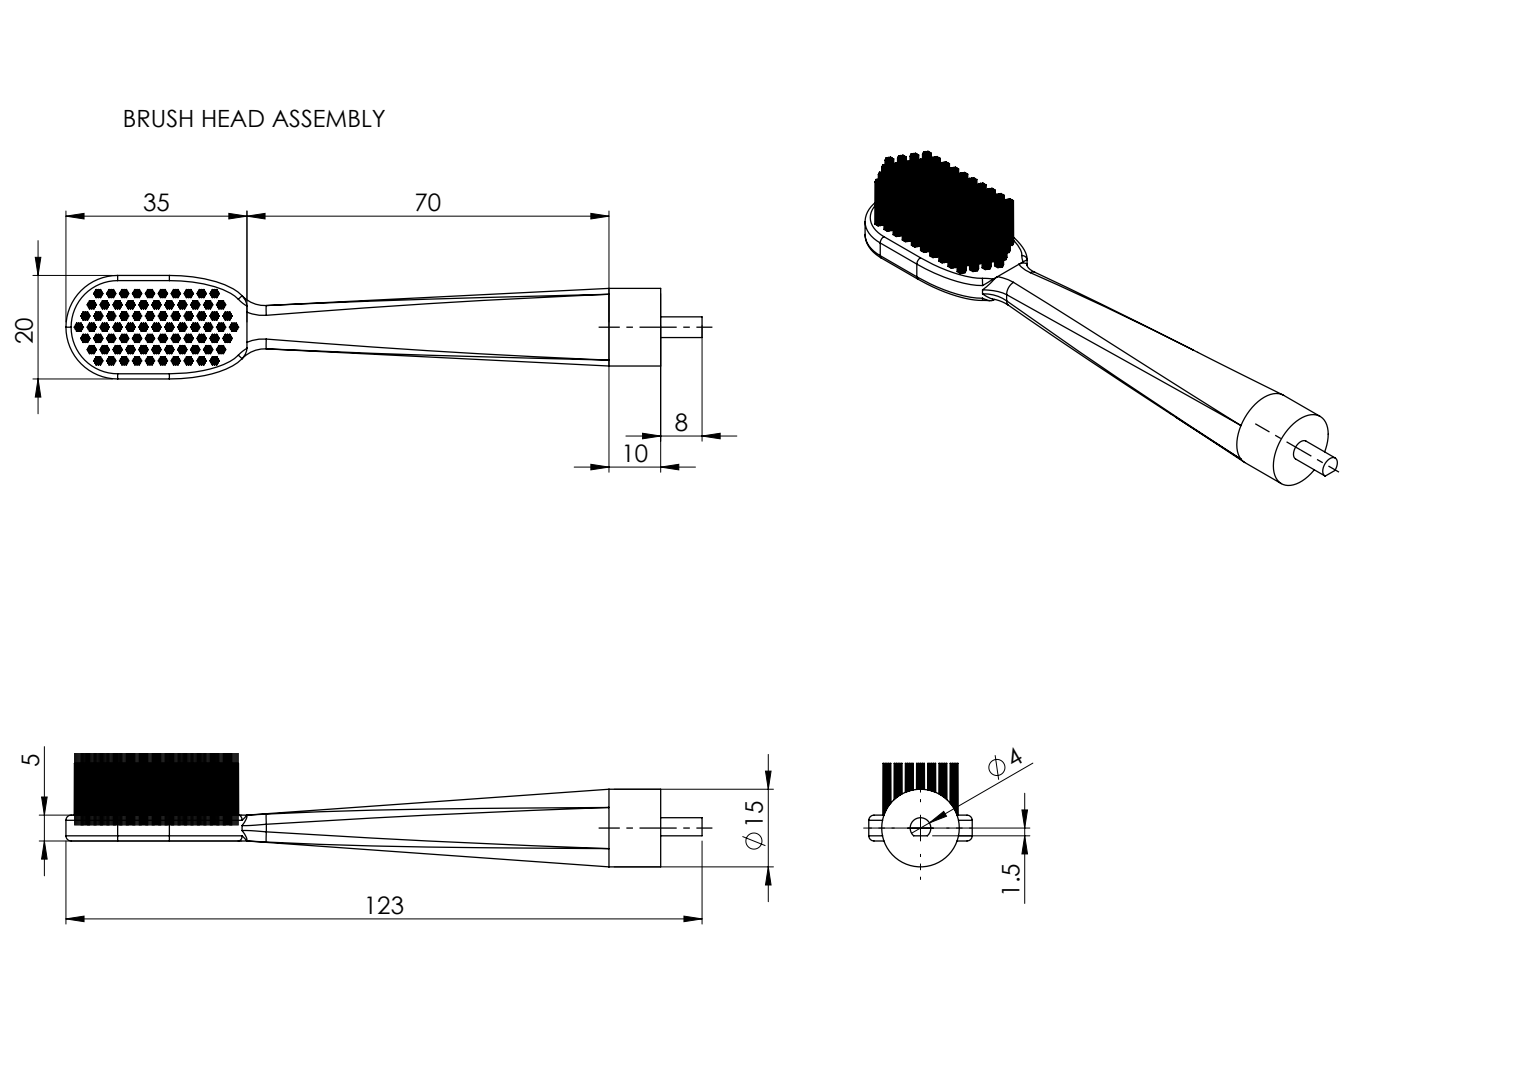
ISO-10303-21;
HEADER;
FILE_DESCRIPTION (('STEP AP214'),
    '1' );
FILE_NAME ('Brush Head Assembly.step',
    '2026-10-02T09:26:43',
    ( '' ),
    ( '' ),
    'SwSTEP 2.0',
    'SolidWorks 2026',
    '' );
FILE_SCHEMA (( 'AUTOMOTIVE_DESIGN' ));
ENDSEC;

DATA;
#1=ORIENTED_EDGE ( 'NONE', *, *, #111289, .F. ) ;
#2=FACE_OUTER_BOUND ( 'NONE', #57861, .T. ) ;
#3=DIRECTION ( 'NONE',  ( 0.000000000000000000, -0.000000000000000000, 1.000000000000000000 ) ) ;
#4=EDGE_CURVE ( 'NONE', #10582, #102432, #129340, .T. ) ;
#6=CIRCLE ( 'NONE', #73182, 0.09999999999999982514 ) ;
#7=CARTESIAN_POINT ( 'NONE',  ( -5.200000000000025935, 12.50000000000000000, -3.983716857408426293 ) ) ;
#8=ADVANCED_FACE ( 'NONE', ( #9369 ), #58491, .T. ) ;
#9=ORIENTED_EDGE ( 'NONE', *, *, #43622, .T. ) ;
#10=DIRECTION ( 'NONE',  ( -0.000000000000000000, 1.000000000000000000, -0.000000000000000000 ) ) ;
#11=AXIS2_PLACEMENT_3D ( 'NONE', #114880, #25207, #65127 ) ;
#12=AXIS2_PLACEMENT_3D ( 'NONE', #43008, #33796, #72443 ) ;
#13=DIRECTION ( 'NONE',  ( 0.000000000000000000, 1.000000000000000000, 0.000000000000000000 ) ) ;
#14=DIRECTION ( 'NONE',  ( 0.000000000000000000, 1.000000000000000000, 0.000000000000000000 ) ) ;
#15=DIRECTION ( 'NONE',  ( 0.000000000000000000, 0.000000000000000000, 1.000000000000000000 ) ) ;
#16=ORIENTED_EDGE ( 'NONE', *, *, #85327, .F. ) ;
#17=ADVANCED_FACE ( 'NONE', ( #79412 ), #68276, .T. ) ;
#18=ORIENTED_EDGE ( 'NONE', *, *, #72941, .T. ) ;
#19=EDGE_CURVE ( 'NONE', #47255, #7520, #102130, .T. ) ;
#20=LINE ( 'NONE', #41902, #103658 ) ;
#21=ORIENTED_EDGE ( 'NONE', *, *, #108659, .T. ) ;
#22=DIRECTION ( 'NONE',  ( 0.000000000000000000, -0.000000000000000000, 1.000000000000000000 ) ) ;
#23=AXIS2_PLACEMENT_3D ( 'NONE', #13282, #3477, #97012 ) ;
#24=CIRCLE ( 'NONE', #104488, 0.1000000000000002554 ) ;
#25=CARTESIAN_POINT ( 'NONE',  ( 17.50000000000000000, -2.499999999999999556, 2.333333333333337478 ) ) ;
#26=DIRECTION ( 'NONE',  ( -0.000000000000000000, -1.000000000000000000, -0.000000000000000000 ) ) ;
#27=VERTEX_POINT ( 'NONE', #38865 ) ;
#28=EDGE_CURVE ( 'NONE', #7615, #17965, #5955, .T. ) ;
#29=CARTESIAN_POINT ( 'NONE',  ( -3.350000000000028511, 2.500000000000000000, -1.472243186433550122 ) ) ;
#30=CARTESIAN_POINT ( 'NONE',  ( 4.549999999999939426, 2.500000000000000000, -6.495190528383302464 ) ) ;
#31=DIRECTION ( 'NONE',  ( 0.000000000000000000, 0.000000000000000000, 1.000000000000000000 ) ) ;
#33=DIRECTION ( 'NONE',  ( 0.000000000000000000, -0.000000000000000000, 1.000000000000000000 ) ) ;
#34=EDGE_CURVE ( 'NONE', #123793, #101138, #123060, .T. ) ;
#35=DIRECTION ( 'NONE',  ( 0.000000000000000000, 0.000000000000000000, 1.000000000000000000 ) ) ;
#36=EDGE_LOOP ( 'NONE', ( #12557, #1627 ) ) ;
#37=ORIENTED_EDGE ( 'NONE', *, *, #25424, .T. ) ;
#38=CARTESIAN_POINT ( 'NONE',  ( -12.09999999999999609, 12.50000000000000000, -3.637306695894647390 ) ) ;
#39=ORIENTED_EDGE ( 'NONE', *, *, #32172, .F. ) ;
#40=DIRECTION ( 'NONE',  ( -0.000000000000000000, 1.000000000000000000, -0.000000000000000000 ) ) ;
#41=ORIENTED_EDGE ( 'NONE', *, *, #63489, .F. ) ;
#42=ORIENTED_EDGE ( 'NONE', *, *, #56795, .T. ) ;
#43=ORIENTED_EDGE ( 'NONE', *, *, #113565, .F. ) ;
#44=CARTESIAN_POINT ( 'NONE',  ( 87.49999999999998579, 2.781865847474100040, -7.000342182495692178 ) ) ;
#45=CIRCLE ( 'NONE', #54416, 0.09999999999999982514 ) ;
#46=CARTESIAN_POINT ( 'NONE',  ( -4.150000000000027889, 12.50000000000000000, -7.253104124594891289 ) ) ;
#47=AXIS2_PLACEMENT_3D ( 'NONE', #50299, #49672, #91507 ) ;
#48=CARTESIAN_POINT ( 'NONE',  ( 10.44999999999991047, 2.500000000000000000, 2.065063509461097624 ) ) ;
#49=CARTESIAN_POINT ( 'NONE',  ( -7.300000000000018474, 12.50000000000000000, 0.3464101615137735735 ) ) ;
#50=DIRECTION ( 'NONE',  ( 0.000000000000000000, -1.000000000000000000, 0.000000000000000000 ) ) ;
#51=DIRECTION ( 'NONE',  ( 0.000000000000000000, 1.000000000000000000, 0.000000000000000000 ) ) ;
#52=CARTESIAN_POINT ( 'NONE',  ( 5.649999999999932854, 2.500000000000000000, 1.918653347947321564 ) ) ;
#53=DIRECTION ( 'NONE',  ( 0.000000000000000000, 0.000000000000000000, 1.000000000000000000 ) ) ;
#54=FACE_OUTER_BOUND ( 'NONE', #43393, .T. ) ;
#55=AXIS2_PLACEMENT_3D ( 'NONE', #102666, #47947, #87846 ) ;
#56=ORIENTED_EDGE ( 'NONE', *, *, #30639, .F. ) ;
#57=ORIENTED_EDGE ( 'NONE', *, *, #57612, .F. ) ;
#58=DIRECTION ( 'NONE',  ( 0.000000000000000000, 0.000000000000000000, -1.000000000000000000 ) ) ;
#59=EDGE_LOOP ( 'NONE', ( #8980, #73677, #9720, #73966 ) ) ;
#60=EDGE_LOOP ( 'NONE', ( #125831, #14201 ) ) ;
#62=CIRCLE ( 'NONE', #54353, 0.09999999999999982514 ) ;
#63=EDGE_CURVE ( 'NONE', #31481, #67997, #18539, .T. ) ;
#64=AXIS2_PLACEMENT_3D ( 'NONE', #6513, #46469, #75933 ) ;
#66=CIRCLE ( 'NONE', #71172, 0.09999999999999982514 ) ;
#67=DIRECTION ( 'NONE',  ( -4.274815082592931898E-19, -0.9999939076577903929, -0.003490651415223739937 ) ) ;
#68=PLANE ( 'NONE',  #922 ) ;
#69=ADVANCED_FACE ( 'NONE', ( #17890 ), #95870, .T. ) ;
#70=DIRECTION ( 'NONE',  ( 0.000000000000000000, -0.9999939076577903929, 0.003490651415223739937 ) ) ;
#71=ORIENTED_EDGE ( 'NONE', *, *, #16257, .F. ) ;
#72=EDGE_CURVE ( 'NONE', #118132, #124753, #125105, .T. ) ;
#73=EDGE_CURVE ( 'NONE', #114203, #127721, #49320, .T. ) ;
#74=AXIS2_PLACEMENT_3D ( 'NONE', #92885, #52954, #31387 ) ;
#75=ADVANCED_FACE ( 'NONE', ( #29656 ), #54076, .T. ) ;
#76=VERTEX_POINT ( 'NONE', #89217 ) ;
#77=PLANE ( 'NONE',  #104864 ) ;
#78=EDGE_LOOP ( 'NONE', ( #93082, #10412 ) ) ;
#79=CARTESIAN_POINT ( 'NONE',  ( 3.549999999999941203, 2.500000000000000000, 6.248780366869521430 ) ) ;
#80=EDGE_CURVE ( 'NONE', #111625, #116591, #38188, .T. ) ;
#81=AXIS2_PLACEMENT_3D ( 'NONE', #66786, #108010, #119130 ) ;
#82=ORIENTED_EDGE ( 'NONE', *, *, #37576, .T. ) ;
#83=ORIENTED_EDGE ( 'NONE', *, *, #49852, .F. ) ;
#84=DIRECTION ( 'NONE',  ( -0.000000000000000000, 1.000000000000000000, -0.000000000000000000 ) ) ;
#85=CARTESIAN_POINT ( 'NONE',  ( -7.100000000000017408, 2.500000000000000000, -4.922947341949753586 ) ) ;
#86=EDGE_CURVE ( 'NONE', #7115, #38409, #127252, .T. ) ;
#87=ADVANCED_FACE ( 'NONE', ( #57833 ), #118026, .T. ) ;
#88=CARTESIAN_POINT ( 'NONE',  ( 13.34999999999990017, 2.500000000000000000, 1.572243186433545548 ) ) ;
#89=DIRECTION ( 'NONE',  ( 0.000000000000000000, 0.000000000000000000, 1.000000000000000000 ) ) ;
#90=CARTESIAN_POINT ( 'NONE',  ( 17.50000000000000000, -2.083333333333333925, 4.000000000000001776 ) ) ;
#91=ORIENTED_EDGE ( 'NONE', *, *, #128566, .T. ) ;
#93=DIRECTION ( 'NONE',  ( -0.000000000000000000, 1.000000000000000000, -0.000000000000000000 ) ) ;
#94=DIRECTION ( 'NONE',  ( -4.274815082592931898E-19, -0.9999939076577903929, -0.003490651415223739937 ) ) ;
#95=CARTESIAN_POINT ( 'NONE',  ( -2.050000000000033129, 2.500000000000000000, 2.165063509461097713 ) ) ;
#96=CARTESIAN_POINT ( 'NONE',  ( -2.950000000000029932, 2.500000000000000000, -2.165063509461101710 ) ) ;
#97=FACE_OUTER_BOUND ( 'NONE', #13668, .T. ) ;
#98=EDGE_LOOP ( 'NONE', ( #5007, #26491, #107521, #16284 ) ) ;
#99=ORIENTED_EDGE ( 'NONE', *, *, #48484, .T. ) ;
#100=CIRCLE ( 'NONE', #16803, 0.06509327318403745899 ) ;
#101=DIRECTION ( 'NONE',  ( 0.000000000000000000, -0.000000000000000000, 1.000000000000000000 ) ) ;
#102=AXIS2_PLACEMENT_3D ( 'NONE', #59335, #77010, #59983 ) ;
#103=ORIENTED_EDGE ( 'NONE', *, *, #8467, .T. ) ;
#104=CARTESIAN_POINT ( 'NONE',  ( 17.41716098457700923, -1.872967139268051806, 4.643356076170615410 ) ) ;
#105=LINE ( 'NONE', #118591, #98263 ) ;
#106=AXIS2_PLACEMENT_3D ( 'NONE', #112814, #42811, #102353 ) ;
#107=VERTEX_POINT ( 'NONE', #106909 ) ;
#108=DIRECTION ( 'NONE',  ( 0.000000000000000000, 1.000000000000000000, 0.000000000000000000 ) ) ;
#109=CARTESIAN_POINT ( 'NONE',  ( -6.650000000000019007, 2.500000000000000000, -5.802370205355749988 ) ) ;
#110=CARTESIAN_POINT ( 'NONE',  ( 10.39999999999991509, 12.50000000000000000, -0.6928203230275542523 ) ) ;
#112=FACE_OUTER_BOUND ( 'NONE', #22375, .T. ) ;
#113=VERTEX_POINT ( 'NONE', #17219 ) ;
#114=DIRECTION ( 'NONE',  ( 0.000000000000000000, -0.9999939076577903929, 0.003490651415223739937 ) ) ;
#115=DIRECTION ( 'NONE',  ( 0.000000000000000000, 0.000000000000000000, 1.000000000000000000 ) ) ;
#116=CARTESIAN_POINT ( 'NONE',  ( -5.200000000000022382, 12.50000000000000000, 0.2813168883297361700 ) ) ;
#117=ADVANCED_FACE ( 'NONE', ( #57173 ), #7419, .T. ) ;
#118=VERTEX_POINT ( 'NONE', #50574 ) ;
#119=DIRECTION ( 'NONE',  ( -0.000000000000000000, 1.000000000000000000, -0.000000000000000000 ) ) ;
#120=EDGE_LOOP ( 'NONE', ( #58165, #15953, #18369, #114695 ) ) ;
#122=DIRECTION ( 'NONE',  ( 0.000000000000000000, -0.000000000000000000, 1.000000000000000000 ) ) ;
#123=DIRECTION ( 'NONE',  ( -4.274815082592931898E-19, -0.9999939076577903929, -0.003490651415223739937 ) ) ;
#124=VERTEX_POINT ( 'NONE', #122556 ) ;
#125=VECTOR ( 'NONE', #104094, 1000.000000000000000 ) ;
#126=CARTESIAN_POINT ( 'NONE',  ( 2.099999999999950351, 12.50000000000000000, -5.022947341949754119 ) ) ;
#127=CONICAL_SURFACE ( 'NONE', #108793, 0.1000000000000000472, 0.003490658503988666988 ) ;
#128=CARTESIAN_POINT ( 'NONE',  ( 1.449999999999951328, 12.50000000000000000, -1.883746621131363597 ) ) ;
#129=EDGE_LOOP ( 'NONE', ( #126937, #8373, #2231, #124616 ) ) ;
#130=CARTESIAN_POINT ( 'NONE',  ( 8.749999999999957367, 2.500000000000000000, -6.595190528383302109 ) ) ;
#131=EDGE_LOOP ( 'NONE', ( #50533, #103161, #4898, #53969 ) ) ;
#132=CONICAL_SURFACE ( 'NONE', #108799, 0.1000000000000002554, 0.003490658503988666988 ) ;
#133=FACE_OUTER_BOUND ( 'NONE', #40974, .T. ) ;
#134=ORIENTED_EDGE ( 'NONE', *, *, #111458, .F. ) ;
#135=DIRECTION ( 'NONE',  ( 0.000000000000000000, 0.000000000000000000, 1.000000000000000000 ) ) ;
#136=CARTESIAN_POINT ( 'NONE',  ( -5.000000000000023093, 2.500000000000000000, 5.022947341949748790 ) ) ;
#137=VERTEX_POINT ( 'NONE', #41429 ) ;
#138=ORIENTED_EDGE ( 'NONE', *, *, #94725, .F. ) ;
#139=DIRECTION ( 'NONE',  ( -0.000000000000000000, 1.000000000000000000, -0.000000000000000000 ) ) ;
#141=ORIENTED_EDGE ( 'NONE', *, *, #10108, .F. ) ;
#142=AXIS2_PLACEMENT_3D ( 'NONE', #9136, #110553, #47778 ) ;
#143=FACE_OUTER_BOUND ( 'NONE', #8076, .T. ) ;
#145=AXIS2_PLACEMENT_3D ( 'NONE', #45558, #95932, #15417 ) ;
#146=DIRECTION ( 'NONE',  ( 0.000000000000000000, 0.000000000000000000, 1.000000000000000000 ) ) ;
#147=CARTESIAN_POINT ( 'NONE',  ( -13.94999999999998685, 12.50000000000000000, -2.576566944158912964 ) ) ;
#148=CARTESIAN_POINT ( 'NONE',  ( -8.300000000000009592, 12.50000000000000000, 4.395220292106234439 ) ) ;
#149=DIRECTION ( 'NONE',  ( 0.000000000000000000, 0.000000000000000000, -1.000000000000000000 ) ) ;
#150=CARTESIAN_POINT ( 'NONE',  ( -0.6500000000000394351, 2.500000000000000000, 6.941600689897073018 ) ) ;
#151=CONICAL_SURFACE ( 'NONE', #75377, 0.09999999999999982514, 0.003490658503988666988 ) ;
#152=EDGE_CURVE ( 'NONE', #35689, #125708, #77064, .T. ) ;
#153=ORIENTED_EDGE ( 'NONE', *, *, #4789, .F. ) ;
#154=ORIENTED_EDGE ( 'NONE', *, *, #109368, .T. ) ;
#155=ORIENTED_EDGE ( 'NONE', *, *, #127999, .F. ) ;
#156=AXIS2_PLACEMENT_3D ( 'NONE', #115565, #16713, #35116 ) ;
#157=CARTESIAN_POINT ( 'NONE',  ( -6.249999999999981348, 12.50000000000000000, 2.165063509461097713 ) ) ;
#158=DIRECTION ( 'NONE',  ( -0.000000000000000000, 1.000000000000000000, -0.000000000000000000 ) ) ;
#159=DIRECTION ( 'NONE',  ( 0.000000000000000000, 0.000000000000000000, 1.000000000000000000 ) ) ;
#160=EDGE_LOOP ( 'NONE', ( #92531, #41100 ) ) ;
#161=EDGE_CURVE ( 'NONE', #53677, #62914, #60358, .T. ) ;
#162=FACE_BOUND ( 'NONE', #99510, .T. ) ;
#163=ORIENTED_EDGE ( 'NONE', *, *, #63007, .F. ) ;
#164=EDGE_CURVE ( 'NONE', #64447, #41921, #37367, .T. ) ;
#165=CARTESIAN_POINT ( 'NONE',  ( -7.900000000000014566, 12.50000000000000000, 0.6277270498435120194 ) ) ;
#166=CARTESIAN_POINT ( 'NONE',  ( 7.899999999999924860, 2.500000000000000000, 5.022947341949748790 ) ) ;
#167=LINE ( 'NONE', #110140, #49263 ) ;
#168=FACE_OUTER_BOUND ( 'NONE', #42884, .T. ) ;
#169=DIRECTION ( 'NONE',  ( -0.000000000000000000, 1.000000000000000000, -0.000000000000000000 ) ) ;
#170=EDGE_CURVE ( 'NONE', #109777, #63696, #31113, .T. ) ;
#171=DIRECTION ( 'NONE',  ( 0.000000000000000000, 1.000000000000000000, 0.000000000000000000 ) ) ;
#172=EDGE_CURVE ( 'NONE', #110736, #16781, #3893, .T. ) ;
#173=DIRECTION ( 'NONE',  ( 0.000000000000000000, 0.000000000000000000, -1.000000000000000000 ) ) ;
#174=EDGE_CURVE ( 'NONE', #53227, #49994, #90490, .T. ) ;
#175=CARTESIAN_POINT ( 'NONE',  ( 11.84999999999990727, 2.500000000000000000, 6.841600689897072485 ) ) ;
#176=ADVANCED_FACE ( 'NONE', ( #101629 ), #14347, .T. ) ;
#177=FACE_OUTER_BOUND ( 'NONE', #72478, .T. ) ;
#178=ORIENTED_EDGE ( 'NONE', *, *, #7339, .F. ) ;
#179=VERTEX_POINT ( 'NONE', #111417 ) ;
#180=VERTEX_POINT ( 'NONE', #20488 ) ;
#181=VERTEX_POINT ( 'NONE', #62977 ) ;
#182=DIRECTION ( 'NONE',  ( 0.000000000000000000, 1.000000000000000000, 0.000000000000000000 ) ) ;
#183=CIRCLE ( 'NONE', #48229, 0.06509327318403741736 ) ;
#184=LINE ( 'NONE', #92445, #36085 ) ;
#185=AXIS2_PLACEMENT_3D ( 'NONE', #74145, #15849, #15191 ) ;
#186=AXIS2_PLACEMENT_3D ( 'NONE', #87460, #107759, #127405 ) ;
#187=EDGE_LOOP ( 'NONE', ( #105520, #67716, #77716, #43576 ) ) ;
#188=ORIENTED_EDGE ( 'NONE', *, *, #84597, .T. ) ;
#189=EDGE_CURVE ( 'NONE', #19176, #5233, #120978, .T. ) ;
#190=ORIENTED_EDGE ( 'NONE', *, *, #82832, .T. ) ;
#191=AXIS2_PLACEMENT_3D ( 'NONE', #50501, #49243, #90414 ) ;
#192=DIRECTION ( 'NONE',  ( -0.000000000000000000, -1.000000000000000000, -0.000000000000000000 ) ) ;
#193=DIRECTION ( 'NONE',  ( 0.000000000000000000, -0.000000000000000000, 1.000000000000000000 ) ) ;
#194=DIRECTION ( 'NONE',  ( -0.000000000000000000, -1.000000000000000000, -0.000000000000000000 ) ) ;
#195=DIRECTION ( 'NONE',  ( 0.000000000000000000, 0.000000000000000000, -1.000000000000000000 ) ) ;
#196=CARTESIAN_POINT ( 'NONE',  ( -8.950000000000004619, 12.50000000000000000, 6.148780366869520897 ) ) ;
#197=CONICAL_SURFACE ( 'NONE', #119337, 0.1000000000000000056, 0.003490658503988666988 ) ;
#198=DIRECTION ( 'NONE',  ( 0.000000000000000000, -0.000000000000000000, 1.000000000000000000 ) ) ;
#199=ORIENTED_EDGE ( 'NONE', *, *, #119327, .F. ) ;
#200=DIRECTION ( 'NONE',  ( 0.000000000000000000, -0.9999939076577903929, 0.003490651415223739937 ) ) ;
#201=ORIENTED_EDGE ( 'NONE', *, *, #13341, .F. ) ;
#202=ORIENTED_EDGE ( 'NONE', *, *, #70316, .F. ) ;
#203=ORIENTED_EDGE ( 'NONE', *, *, #126845, .T. ) ;
#204=DIRECTION ( 'NONE',  ( -0.000000000000000000, -1.000000000000000000, -0.000000000000000000 ) ) ;
#205=EDGE_CURVE ( 'NONE', #70284, #50485, #21114, .T. ) ;
#206=ORIENTED_EDGE ( 'NONE', *, *, #92160, .F. ) ;
#207=ORIENTED_EDGE ( 'NONE', *, *, #83833, .F. ) ;
#209=AXIS2_PLACEMENT_3D ( 'NONE', #67296, #8398, #18868 ) ;
#210=CARTESIAN_POINT ( 'NONE',  ( 9.399999999999915090, 2.500000000000000000, 3.983716857408420964 ) ) ;
#211=CARTESIAN_POINT ( 'NONE',  ( 14.14999999999989377, 2.500000000000000000, -2.857883832488653741 ) ) ;
#212=DIRECTION ( 'NONE',  ( -0.000000000000000000, 1.000000000000000000, -0.000000000000000000 ) ) ;
#213=ADVANCED_FACE ( 'NONE', ( #70872 ), #100964, .T. ) ;
#214=DIRECTION ( 'NONE',  ( -0.000000000000000000, 1.000000000000000000, -0.000000000000000000 ) ) ;
#215=EDGE_CURVE ( 'NONE', #14404, #106677, #98609, .T. ) ;
#218=DIRECTION ( 'NONE',  ( 0.000000000000000000, 1.000000000000000000, 0.000000000000000000 ) ) ;
#219=CONICAL_SURFACE ( 'NONE', #115215, 0.1000000000000000472, 0.003490658503988666988 ) ;
#220=CIRCLE ( 'NONE', #73386, 0.06509327318403745899 ) ;
#221=ORIENTED_EDGE ( 'NONE', *, *, #31291, .F. ) ;
#222=DIRECTION ( 'NONE',  ( 0.000000000000000000, 0.000000000000000000, 1.000000000000000000 ) ) ;
#224=VERTEX_POINT ( 'NONE', #112735 ) ;
#225=DIRECTION ( 'NONE',  ( -0.000000000000000000, 1.000000000000000000, -0.000000000000000000 ) ) ;
#226=CARTESIAN_POINT ( 'NONE',  ( 21.24754738303297330, 0.7337760880902002292, -4.182111650399407132 ) ) ;
#227=ADVANCED_FACE ( 'NONE', ( #89853 ), #30320, .T. ) ;
#228=ORIENTED_EDGE ( 'NONE', *, *, #115605, .T. ) ;
#229=CARTESIAN_POINT ( 'NONE',  ( 5.599999999999931255, 12.50000000000000000, 3.918623584224382839 ) ) ;
#230=EDGE_CURVE ( 'NONE', #34015, #92739, #32256, .T. ) ;
#231=DIRECTION ( 'NONE',  ( 0.000000000000000000, 0.000000000000000000, -1.000000000000000000 ) ) ;
#232=EDGE_LOOP ( 'NONE', ( #14783, #39929, #121308, #33112 ) ) ;
#233=CONICAL_SURFACE ( 'NONE', #8535, 0.1000000000000002554, 0.003490658503988666988 ) ;
#234=EDGE_CURVE ( 'NONE', #45310, #78495, #22435, .T. ) ;
#235=AXIS2_PLACEMENT_3D ( 'NONE', #117904, #58371, #98266 ) ;
#236=EDGE_CURVE ( 'NONE', #86441, #35274, #92360, .T. ) ;
#237=EDGE_CURVE ( 'NONE', #3662, #62906, #43359, .T. ) ;
#238=CARTESIAN_POINT ( 'NONE',  ( 10.64999999999990976, 12.50000000000000000, 1.753560074763284016 ) ) ;
#239=ORIENTED_EDGE ( 'NONE', *, *, #20618, .F. ) ;
#241=DIRECTION ( 'NONE',  ( 0.000000000000000000, 0.000000000000000000, 1.000000000000000000 ) ) ;
#242=FACE_OUTER_BOUND ( 'NONE', #74937, .T. ) ;
#243=LINE ( 'NONE', #68992, #50135 ) ;
#244=DIRECTION ( 'NONE',  ( 0.000000000000000000, 0.000000000000000000, 1.000000000000000000 ) ) ;
#246=AXIS2_PLACEMENT_3D ( 'NONE', #45056, #45692, #64672 ) ;
#247=CIRCLE ( 'NONE', #62948, 0.1000000000000000472 ) ;
#248=CARTESIAN_POINT ( 'NONE',  ( 6.049999999999935874, 2.500000000000000000, -6.941600689897077459 ) ) ;
#249=VERTEX_POINT ( 'NONE', #105488 ) ;
#250=DIRECTION ( 'NONE',  ( -0.000000000000000000, -1.000000000000000000, -0.000000000000000000 ) ) ;
#251=VERTEX_POINT ( 'NONE', #124483 ) ;
#252=CARTESIAN_POINT ( 'NONE',  ( -1.450000000000035483, 12.50000000000000000, 1.883746621131358934 ) ) ;
#253=CARTESIAN_POINT ( 'NONE',  ( 8.099999999999921485, 2.500000000000000000, 0.2464101615137735679 ) ) ;
#254=AXIS2_PLACEMENT_3D ( 'NONE', #24478, #34962, #47347 ) ;
#255=AXIS2_PLACEMENT_3D ( 'NONE', #22150, #12292, #81057 ) ;
#257=PLANE ( 'NONE',  #99050 ) ;
#258=DIRECTION ( 'NONE',  ( 0.000000000000000000, -0.9999939076577903929, 0.003490651415223739937 ) ) ;
#259=DIRECTION ( 'NONE',  ( 0.000000000000000000, 0.000000000000000000, 1.000000000000000000 ) ) ;
#260=CARTESIAN_POINT ( 'NONE',  ( -11.89999999999999680, 2.500000000000000000, -4.576537180435975571 ) ) ;
#261=ORIENTED_EDGE ( 'NONE', *, *, #25908, .F. ) ;
#262=DIRECTION ( 'NONE',  ( 0.000000000000000000, -0.9999939076577903929, 0.003490651415223739937 ) ) ;
#263=DIRECTION ( 'NONE',  ( -0.000000000000000000, 1.000000000000000000, -0.000000000000000000 ) ) ;
#264=CARTESIAN_POINT ( 'NONE',  ( 13.14999999999989733, 2.500000000000000000, -2.511473670974877948 ) ) ;
#265=ORIENTED_EDGE ( 'NONE', *, *, #80354, .F. ) ;
#266=CARTESIAN_POINT ( 'NONE',  ( -11.44999999999999929, 2.500000000000000000, -1.718653347947322052 ) ) ;
#267=EDGE_CURVE ( 'NONE', #13125, #47712, #71425, .T. ) ;
#268=EDGE_LOOP ( 'NONE', ( #106768, #28625 ) ) ;
#269=VERTEX_POINT ( 'NONE', #123201 ) ;
#270=DIRECTION ( 'NONE',  ( 0.000000000000000000, 0.000000000000000000, 1.000000000000000000 ) ) ;
#271=AXIS2_PLACEMENT_3D ( 'NONE', #106645, #15669, #35977 ) ;
#272=AXIS2_PLACEMENT_3D ( 'NONE', #94108, #74472, #114381 ) ;
#273=AXIS2_PLACEMENT_3D ( 'NONE', #118714, #118066, #68969 ) ;
#274=EDGE_LOOP ( 'NONE', ( #97297, #118927 ) ) ;
#275=DIRECTION ( 'NONE',  ( 0.000000000000000000, 0.000000000000000000, 1.000000000000000000 ) ) ;
#276=CARTESIAN_POINT ( 'NONE',  ( 5.799999999999931433, 12.50000000000000000, 4.395220292106234439 ) ) ;
#277=ORIENTED_EDGE ( 'NONE', *, *, #87516, .F. ) ;
#278=VECTOR ( 'NONE', #38628, 1000.000000000000000 ) ;
#279=LINE ( 'NONE', #110252, #23714 ) ;
#280=CIRCLE ( 'NONE', #81853, 0.06509327318403741736 ) ;
#281=DIRECTION ( 'NONE',  ( 0.000000000000000000, -0.9999939076577903929, 0.003490651415223739937 ) ) ;
#282=DIRECTION ( 'NONE',  ( 0.000000000000000000, 0.000000000000000000, 1.000000000000000000 ) ) ;
#283=ADVANCED_FACE ( 'NONE', ( #24987 ), #65155, .T. ) ;
#284=ORIENTED_EDGE ( 'NONE', *, *, #126777, .T. ) ;
#285=ORIENTED_EDGE ( 'NONE', *, *, #2427, .F. ) ;
#286=ORIENTED_EDGE ( 'NONE', *, *, #35114, .F. ) ;
#287=DIRECTION ( 'NONE',  ( -0.000000000000000000, -1.000000000000000000, -0.000000000000000000 ) ) ;
#288=DIRECTION ( 'NONE',  ( 0.000000000000000000, 0.000000000000000000, 1.000000000000000000 ) ) ;
#289=DIRECTION ( 'NONE',  ( -0.000000000000000000, 1.000000000000000000, -0.000000000000000000 ) ) ;
#290=FACE_BOUND ( 'NONE', #126554, .T. ) ;
#291=ORIENTED_EDGE ( 'NONE', *, *, #83216, .F. ) ;
#292=DIRECTION ( 'NONE',  ( 0.000000000000000000, 0.000000000000000000, 1.000000000000000000 ) ) ;
#293=DIRECTION ( 'NONE',  ( 0.000000000000000000, -0.000000000000000000, 1.000000000000000000 ) ) ;
#294=ORIENTED_EDGE ( 'NONE', *, *, #21313, .F. ) ;
#295=DIRECTION ( 'NONE',  ( 0.000000000000000000, 0.000000000000000000, -1.000000000000000000 ) ) ;
#296=CARTESIAN_POINT ( 'NONE',  ( -11.04999999999999893, 2.500000000000000000, 1.818653347947321475 ) ) ;
#297=DIRECTION ( 'NONE',  ( -0.000000000000000000, -1.000000000000000000, -0.000000000000000000 ) ) ;
#298=DIRECTION ( 'NONE',  ( 0.000000000000000000, -0.9999939076577903929, 0.003490651415223739937 ) ) ;
#299=CARTESIAN_POINT ( 'NONE',  ( 2.049999999999950084, 2.500000000000000000, 2.165063509461097713 ) ) ;
#300=DIRECTION ( 'NONE',  ( 0.000000000000000000, 1.000000000000000000, 0.000000000000000000 ) ) ;
#301=LINE ( 'NONE', #128666, #48207 ) ;
#302=CIRCLE ( 'NONE', #73475, 0.1000000000000000472 ) ;
#303=EDGE_CURVE ( 'NONE', #26935, #23200, #114647, .T. ) ;
#304=ORIENTED_EDGE ( 'NONE', *, *, #29474, .T. ) ;
#305=ORIENTED_EDGE ( 'NONE', *, *, #98641, .F. ) ;
#306=ORIENTED_EDGE ( 'NONE', *, *, #68939, .F. ) ;
#307=EDGE_LOOP ( 'NONE', ( #81864, #53697, #107603, #18782 ) ) ;
#308=DIRECTION ( 'NONE',  ( 0.000000000000000000, -0.9999939076577903929, 0.003490651415223739937 ) ) ;
#309=CARTESIAN_POINT ( 'NONE',  ( 13.74999999999993072, 2.500000000000000000, -2.165063509461101710 ) ) ;
#310=EDGE_LOOP ( 'NONE', ( #57715, #102459 ) ) ;
#311=FACE_BOUND ( 'NONE', #39121, .T. ) ;
#312=ADVANCED_FACE ( 'NONE', ( #15798 ), #25451, .T. ) ;
#313=LINE ( 'NONE', #12086, #37510 ) ;
#314=VECTOR ( 'NONE', #88274, 1000.000000000000000 ) ;
#315=CIRCLE ( 'NONE', #10772, 0.09999999999999982514 ) ;
#316=DIRECTION ( 'NONE',  ( 0.000000000000000000, 0.000000000000000000, 1.000000000000000000 ) ) ;
#317=CARTESIAN_POINT ( 'NONE',  ( 2.949999999999943334, 12.50000000000000000, 6.495190528383297135 ) ) ;
#318=ADVANCED_FACE ( 'NONE', ( #4048 ), #118462, .T. ) ;
#319=FACE_OUTER_BOUND ( 'NONE', #53920, .T. ) ;
#320=EDGE_CURVE ( 'NONE', #39409, #2500, #55733, .T. ) ;
#321=DIRECTION ( 'NONE',  ( 0.000000000000000000, 0.000000000000000000, 1.000000000000000000 ) ) ;
#322=EDGE_CURVE ( 'NONE', #118758, #53470, #49534, .T. ) ;
#323=CARTESIAN_POINT ( 'NONE',  ( -1.050000000000038680, 2.500000000000000000, 6.741600689897071952 ) ) ;
#324=EDGE_CURVE ( 'NONE', #23588, #89858, #112217, .T. ) ;
#325=EDGE_LOOP ( 'NONE', ( #61905, #50116, #33161, #106060 ) ) ;
#326=EDGE_CURVE ( 'NONE', #98580, #67678, #66234, .T. ) ;
#327=AXIS2_PLACEMENT_3D ( 'NONE', #75611, #34437, #106376 ) ;
#328=ORIENTED_EDGE ( 'NONE', *, *, #89775, .T. ) ;
#329=CIRCLE ( 'NONE', #90217, 0.06509327318403745899 ) ;
#330=ORIENTED_EDGE ( 'NONE', *, *, #80772, .F. ) ;
#331=VERTEX_POINT ( 'NONE', #113362 ) ;
#332=ORIENTED_EDGE ( 'NONE', *, *, #4672, .F. ) ;
#333=ORIENTED_EDGE ( 'NONE', *, *, #89472, .T. ) ;
#334=VECTOR ( 'NONE', #40375, 1000.000000000000000 ) ;
#335=DIRECTION ( 'NONE',  ( 0.000000000000000000, 1.000000000000000000, 0.000000000000000000 ) ) ;
#336=DIRECTION ( 'NONE',  ( 0.000000000000000000, 1.000000000000000000, 0.000000000000000000 ) ) ;
#337=ORIENTED_EDGE ( 'NONE', *, *, #87514, .F. ) ;
#338=ADVANCED_FACE ( 'NONE', ( #43998 ), #105950, .T. ) ;
#339=CARTESIAN_POINT ( 'NONE',  ( 11.24999999999990585, 12.50000000000000000, -5.802370205355749988 ) ) ;
#340=AXIS2_PLACEMENT_3D ( 'NONE', #87388, #97223, #127343 ) ;
#341=EDGE_CURVE ( 'NONE', #29920, #106540, #93098, .T. ) ;
#342=EDGE_CURVE ( 'NONE', #41239, #126826, #74090, .T. ) ;
#343=CARTESIAN_POINT ( 'NONE',  ( 7.049999999999928768, 2.500000000000000000, -2.165063509461101710 ) ) ;
#344=CIRCLE ( 'NONE', #48391, 0.06509327318403745899 ) ;
#345=CIRCLE ( 'NONE', #4533, 0.06509327318403745899 ) ;
#347=DIRECTION ( 'NONE',  ( 0.000000000000000000, 0.000000000000000000, 1.000000000000000000 ) ) ;
#348=DIRECTION ( 'NONE',  ( 0.000000000000000000, 1.000000000000000000, 0.000000000000000000 ) ) ;
#349=ORIENTED_EDGE ( 'NONE', *, *, #95079, .T. ) ;
#350=FACE_OUTER_BOUND ( 'NONE', #62832, .T. ) ;
#351=ORIENTED_EDGE ( 'NONE', *, *, #55703, .F. ) ;
#352=ORIENTED_EDGE ( 'NONE', *, *, #90036, .T. ) ;
#353=PLANE ( 'NONE',  #42636 ) ;
#355=DIRECTION ( 'NONE',  ( 0.000000000000000000, 0.000000000000000000, -1.000000000000000000 ) ) ;
#356=VERTEX_POINT ( 'NONE', #26287 ) ;
#357=ORIENTED_EDGE ( 'NONE', *, *, #4257, .F. ) ;
#358=PLANE ( 'NONE',  #73574 ) ;
#359=DIRECTION ( 'NONE',  ( 0.000000000000000000, -0.9999939076577903929, 0.003490651415223739937 ) ) ;
#360=CARTESIAN_POINT ( 'NONE',  ( -9.350000000000004974, 2.500000000000000000, 6.148780366869520897 ) ) ;
#361=VECTOR ( 'NONE', #77259, 1000.000000000000000 ) ;
#362=DIRECTION ( 'NONE',  ( 0.000000000000000000, 0.000000000000000000, -1.000000000000000000 ) ) ;
#363=EDGE_LOOP ( 'NONE', ( #37581, #94874, #128100, #15237 ) ) ;
#364=CONICAL_SURFACE ( 'NONE', #12877, 0.1000000000000002554, 0.003490658503988666988 ) ;
#365=VECTOR ( 'NONE', #93137, 1000.000000000000000 ) ;
#366=CARTESIAN_POINT ( 'NONE',  ( -0.8500000000000395017, 2.500000000000000000, 2.065063509461097624 ) ) ;
#367=EDGE_LOOP ( 'NONE', ( #100670, #104053, #13822, #112020 ) ) ;
#368=LINE ( 'NONE', #39705, #26989 ) ;
#369=AXIS2_PLACEMENT_3D ( 'NONE', #120392, #31376, #29436 ) ;
#370=ORIENTED_EDGE ( 'NONE', *, *, #75435, .F. ) ;
#371=FACE_OUTER_BOUND ( 'NONE', #86248, .T. ) ;
#372=AXIS2_PLACEMENT_3D ( 'NONE', #42902, #31772, #111612 ) ;
#373=CARTESIAN_POINT ( 'NONE',  ( 76.44221964357954846, -3.905139022502750024, 5.869652876108133910 ) ) ;
#374=CARTESIAN_POINT ( 'NONE',  ( 0.3999999999999628852, 2.500000000000000000, 0.6928203230275518099 ) ) ;
#375=AXIS2_PLACEMENT_3D ( 'NONE', #56457, #126503, #46017 ) ;
#376=ADVANCED_FACE ( 'NONE', ( #83896 ), #32815, .T. ) ;
#377=CARTESIAN_POINT ( 'NONE',  ( -6.900000000000019007, 2.500000000000000000, -0.2464101615137783419 ) ) ;
#378=VERTEX_POINT ( 'NONE', #53172 ) ;
#379=VECTOR ( 'NONE', #86112, 1000.000000000000000 ) ;
#380=ADVANCED_FACE ( 'NONE', ( #3414 ), #82983, .T. ) ;
#381=DIRECTION ( 'NONE',  ( 0.000000000000000000, 0.000000000000000000, -1.000000000000000000 ) ) ;
#382=EDGE_CURVE ( 'NONE', #121670, #96705, #103561, .T. ) ;
#383=CARTESIAN_POINT ( 'NONE',  ( -10.84999999999999964, 2.500000000000000000, 7.188010851410848723 ) ) ;
#384=VERTEX_POINT ( 'NONE', #98874 ) ;
#386=ORIENTED_EDGE ( 'NONE', *, *, #106988, .T. ) ;
#387=DIRECTION ( 'NONE',  ( 0.000000000000000000, -0.000000000000000000, 1.000000000000000000 ) ) ;
#388=DIRECTION ( 'NONE',  ( 0.000000000000000000, 0.000000000000000000, 1.000000000000000000 ) ) ;
#389=DIRECTION ( 'NONE',  ( 0.000000000000000000, -0.000000000000000000, 1.000000000000000000 ) ) ;
#390=CARTESIAN_POINT ( 'NONE',  ( -13.29999999999999005, 2.500000000000000000, -4.330127018922198978 ) ) ;
#391=DIRECTION ( 'NONE',  ( 0.000000000000000000, 1.000000000000000000, 0.000000000000000000 ) ) ;
#392=ADVANCED_FACE ( 'NONE', ( #7261 ), #95484, .T. ) ;
#393=DIRECTION ( 'NONE',  ( -0.000000000000000000, 1.000000000000000000, -0.000000000000000000 ) ) ;
#394=DIRECTION ( 'NONE',  ( 0.000000000000000000, 1.000000000000000000, 0.000000000000000000 ) ) ;
#395=CARTESIAN_POINT ( 'NONE',  ( -3.750000000000026201, 2.500000000000000000, 5.802370205355744659 ) ) ;
#397=AXIS2_PLACEMENT_3D ( 'NONE', #46964, #58707, #116961 ) ;
#398=AXIS2_PLACEMENT_3D ( 'NONE', #61758, #101673, #11989 ) ;
#399=ORIENTED_EDGE ( 'NONE', *, *, #91207, .T. ) ;
#400=DIRECTION ( 'NONE',  ( -0.000000000000000000, -1.000000000000000000, -0.000000000000000000 ) ) ;
#401=CARTESIAN_POINT ( 'NONE',  ( -14.14999999999998614, 12.50000000000000000, 1.472243186433549456 ) ) ;
#402=CARTESIAN_POINT ( 'NONE',  ( -12.49999999999999289, 12.50000000000000000, -0.6928203230275500335 ) ) ;
#403=ADVANCED_FACE ( 'NONE', ( #66826 ), #37652, .T. ) ;
#404=DIRECTION ( 'NONE',  ( 0.000000000000000000, 0.000000000000000000, 1.000000000000000000 ) ) ;
#405=CARTESIAN_POINT ( 'NONE',  ( 7.049999999999928768, 2.500000000000000000, 6.495190528383297135 ) ) ;
#406=CIRCLE ( 'NONE', #33873, 0.06509327318403745899 ) ;
#407=AXIS2_PLACEMENT_3D ( 'NONE', #20032, #59980, #99882 ) ;
#408=VERTEX_POINT ( 'NONE', #17726 ) ;
#409=CARTESIAN_POINT ( 'NONE',  ( -7.050000000000013145, 2.500000000000000000, 6.595190528383296780 ) ) ;
#410=CIRCLE ( 'NONE', #42297, 0.06509327318403743123 ) ;
#411=CIRCLE ( 'NONE', #58928, 0.06509327318403745899 ) ;
#412=DIRECTION ( 'NONE',  ( -0.000000000000000000, 1.000000000000000000, -0.000000000000000000 ) ) ;
#413=DIRECTION ( 'NONE',  ( 0.000000000000000000, -0.9999939076577903929, 0.003490651415223739937 ) ) ;
#414=ORIENTED_EDGE ( 'NONE', *, *, #38047, .F. ) ;
#415=EDGE_LOOP ( 'NONE', ( #59433, #27224 ) ) ;
#416=CARTESIAN_POINT ( 'NONE',  ( -12.29999999999999716, 2.500000000000000000, 0.4464101615137776591 ) ) ;
#417=CIRCLE ( 'NONE', #107031, 0.06509327318403745899 ) ;
#418=EDGE_CURVE ( 'NONE', #72177, #71951, #50185, .T. ) ;
#419=ORIENTED_EDGE ( 'NONE', *, *, #57235, .T. ) ;
#420=VECTOR ( 'NONE', #30289, 1000.000000000000000 ) ;
#421=AXIS2_PLACEMENT_3D ( 'NONE', #24378, #102927, #93129 ) ;
#422=ORIENTED_EDGE ( 'NONE', *, *, #20340, .F. ) ;
#423=CIRCLE ( 'NONE', #100772, 0.06509327318403745899 ) ;
#424=FACE_OUTER_BOUND ( 'NONE', #6671, .T. ) ;
#425=AXIS2_PLACEMENT_3D ( 'NONE', #127655, #7217, #37985 ) ;
#426=DIRECTION ( 'NONE',  ( 0.000000000000000000, 0.000000000000000000, 1.000000000000000000 ) ) ;
#427=DIRECTION ( 'NONE',  ( -0.000000000000000000, 1.000000000000000000, -0.000000000000000000 ) ) ;
#428=CARTESIAN_POINT ( 'NONE',  ( 0.1999999999999627909, 12.50000000000000000, 0.2813168883297384459 ) ) ;
#429=ORIENTED_EDGE ( 'NONE', *, *, #31666, .F. ) ;
#430=CIRCLE ( 'NONE', #77706, 0.06509327318403745899 ) ;
#431=FACE_OUTER_BOUND ( 'NONE', #54831, .T. ) ;
#432=ORIENTED_EDGE ( 'NONE', *, *, #72222, .F. ) ;
#433=DIRECTION ( 'NONE',  ( -0.000000000000000000, 1.000000000000000000, -0.000000000000000000 ) ) ;
#434=FACE_OUTER_BOUND ( 'NONE', #53931, .T. ) ;
#435=ADVANCED_FACE ( 'NONE', ( #9210 ), #17059, .T. ) ;
#436=DIRECTION ( 'NONE',  ( -4.274815082592931898E-19, -0.9999939076577903929, -0.003490651415223739937 ) ) ;
#437=ORIENTED_EDGE ( 'NONE', *, *, #120658, .F. ) ;
#438=ORIENTED_EDGE ( 'NONE', *, *, #126436, .T. ) ;
#439=ORIENTED_EDGE ( 'NONE', *, *, #64645, .T. ) ;
#440=EDGE_LOOP ( 'NONE', ( #14150, #118505 ) ) ;
#441=EDGE_LOOP ( 'NONE', ( #46577, #104696, #83589, #8113 ) ) ;
#442=CARTESIAN_POINT ( 'NONE',  ( 12.09999999999990550, 2.500000000000000000, -3.637306695894650055 ) ) ;
#443=CARTESIAN_POINT ( 'NONE',  ( 10.06913504587783947, 2.500000000000000888, 8.158951466337887481 ) ) ;
#444=FACE_OUTER_BOUND ( 'NONE', #25643, .T. ) ;
#445=FACE_BOUND ( 'NONE', #8268, .T. ) ;
#446=CARTESIAN_POINT ( 'NONE',  ( 1.249999999999988454, 12.50000000000000000, -2.165063509461101710 ) ) ;
#448=FACE_OUTER_BOUND ( 'NONE', #12746, .T. ) ;
#449=DIRECTION ( 'NONE',  ( -4.274815082592931898E-19, -0.9999939076577903929, -0.003490651415223739937 ) ) ;
#451=DIRECTION ( 'NONE',  ( 0.000000000000000000, -0.000000000000000000, 1.000000000000000000 ) ) ;
#452=AXIS2_PLACEMENT_3D ( 'NONE', #51765, #22319, #31478 ) ;
#453=DIRECTION ( 'NONE',  ( 0.000000000000000000, 1.000000000000000000, 0.000000000000000000 ) ) ;
#454=CARTESIAN_POINT ( 'NONE',  ( 12.49999999999993605, 2.500000000000000000, 0.09999999999999772959 ) ) ;
#455=VECTOR ( 'NONE', #15572, 1000.000000000000000 ) ;
#456=CIRCLE ( 'NONE', #19547, 0.06509327318403745899 ) ;
#457=LINE ( 'NONE', #62637, #1297 ) ;
#458=CIRCLE ( 'NONE', #33938, 0.06509327318403741736 ) ;
#459=EDGE_CURVE ( 'NONE', #71750, #12146, #88396, .T. ) ;
#460=VERTEX_POINT ( 'NONE', #57679 ) ;
#461=EDGE_LOOP ( 'NONE', ( #33703, #45194, #92447, #104543 ) ) ;
#462=EDGE_LOOP ( 'NONE', ( #129077, #120773 ) ) ;
#463=ORIENTED_EDGE ( 'NONE', *, *, #84900, .F. ) ;
#464=AXIS2_PLACEMENT_3D ( 'NONE', #93258, #125292, #35627 ) ;
#465=DIRECTION ( 'NONE',  ( 0.000000000000000000, 0.000000000000000000, 1.000000000000000000 ) ) ;
#466=AXIS2_PLACEMENT_3D ( 'NONE', #7124, #114506, #105988 ) ;
#467=FACE_OUTER_BOUND ( 'NONE', #87408, .T. ) ;
#468=FACE_BOUND ( 'NONE', #114889, .T. ) ;
#469=CONICAL_SURFACE ( 'NONE', #29740, 0.1000000000000002554, 0.003490658503988666988 ) ;
#470=CARTESIAN_POINT ( 'NONE',  ( -10.65000000000000391, 2.500000000000000000, -6.841600689897075149 ) ) ;
#471=EDGE_CURVE ( 'NONE', #91134, #38338, #8544, .T. ) ;
#472=ORIENTED_EDGE ( 'NONE', *, *, #70105, .F. ) ;
#473=ADVANCED_FACE ( 'NONE', ( #48493 ), #54362, .T. ) ;
#474=DIRECTION ( 'NONE',  ( 0.000000000000000000, 0.000000000000000000, 1.000000000000000000 ) ) ;
#475=CARTESIAN_POINT ( 'NONE',  ( -3.150000000000029221, 12.50000000000000000, -1.753560074763288679 ) ) ;
#476=EDGE_CURVE ( 'NONE', #72177, #24862, #37399, .T. ) ;
#477=DIRECTION ( 'NONE',  ( -0.000000000000000000, -1.000000000000000000, -0.000000000000000000 ) ) ;
#478=ADVANCED_FACE ( 'NONE', ( #128368 ), #106587, .T. ) ;
#479=CARTESIAN_POINT ( 'NONE',  ( 10.64999999999991331, 12.50000000000000000, 6.906693963081109722 ) ) ;
#480=EDGE_CURVE ( 'NONE', #103573, #99701, #89867, .T. ) ;
#481=ORIENTED_EDGE ( 'NONE', *, *, #101011, .F. ) ;
#482=DIRECTION ( 'NONE',  ( 0.000000000000000000, 0.000000000000000000, 1.000000000000000000 ) ) ;
#483=ORIENTED_EDGE ( 'NONE', *, *, #114599, .F. ) ;
#484=ADVANCED_FACE ( 'NONE', ( #29503 ), #71094, .T. ) ;
#485=ORIENTED_EDGE ( 'NONE', *, *, #39680, .F. ) ;
#486=CARTESIAN_POINT ( 'NONE',  ( 5.399999999999932854, 12.50000000000000000, 3.637306695894644726 ) ) ;
#487=EDGE_CURVE ( 'NONE', #113497, #31016, #117032, .T. ) ;
#489=ORIENTED_EDGE ( 'NONE', *, *, #128216, .F. ) ;
#490=EDGE_CURVE ( 'NONE', #118039, #58176, #68770, .T. ) ;
#492=EDGE_CURVE ( 'NONE', #2276, #21005, #49161, .T. ) ;
#493=CIRCLE ( 'NONE', #53038, 0.1000000000000000472 ) ;
#494=CARTESIAN_POINT ( 'NONE',  ( 1.449999999999952660, 2.500000000000000000, -6.841600689897078702 ) ) ;
#495=EDGE_CURVE ( 'NONE', #48344, #7845, #16425, .T. ) ;
#496=DIRECTION ( 'NONE',  ( 0.000000000000000000, -0.000000000000000000, 1.000000000000000000 ) ) ;
#497=CARTESIAN_POINT ( 'NONE',  ( 11.24999999999990941, 2.500000000000000000, -1.472243186433550122 ) ) ;
#498=EDGE_LOOP ( 'NONE', ( #49269, #78172, #39117, #88604 ) ) ;
#499=CARTESIAN_POINT ( 'NONE',  ( -15.59999999999998010, 2.500000000000000000, -0.3464101615137759604 ) ) ;
#500=VECTOR ( 'NONE', #4290, 1000.000000000000000 ) ;
#501=EDGE_CURVE ( 'NONE', #82957, #8340, #106126, .T. ) ;
#502=ORIENTED_EDGE ( 'NONE', *, *, #7892, .F. ) ;
#503=FACE_OUTER_BOUND ( 'NONE', #69667, .T. ) ;
#505=CIRCLE ( 'NONE', #65349, 0.06509327318403745899 ) ;
#506=ORIENTED_EDGE ( 'NONE', *, *, #31543, .F. ) ;
#509=CARTESIAN_POINT ( 'NONE',  ( 9.999999999999912959, 2.500000000000000000, 3.637306695894644726 ) ) ;
#511=FACE_OUTER_BOUND ( 'NONE', #69854, .T. ) ;
#512=DIRECTION ( 'NONE',  ( -0.000000000000000000, -1.000000000000000000, -0.000000000000000000 ) ) ;
#513=DIRECTION ( 'NONE',  ( 0.000000000000000000, -0.9999939076577903929, 0.003490651415223739937 ) ) ;
#514=CONICAL_SURFACE ( 'NONE', #100868, 0.09999999999999982514, 0.003490658503988666988 ) ;
#515=VERTEX_POINT ( 'NONE', #96290 ) ;
#516=ORIENTED_EDGE ( 'NONE', *, *, #84359, .T. ) ;
#517=AXIS2_PLACEMENT_3D ( 'NONE', #98837, #49774, #89033 ) ;
#518=ORIENTED_EDGE ( 'NONE', *, *, #80415, .T. ) ;
#519=DIRECTION ( 'NONE',  ( -0.000000000000000000, -1.000000000000000000, -0.000000000000000000 ) ) ;
#520=CARTESIAN_POINT ( 'NONE',  ( -13.74999999999995381, 12.50000000000000000, 2.230156782645138946 ) ) ;
#521=AXIS2_PLACEMENT_3D ( 'NONE', #75882, #85700, #76540 ) ;
#522=CONICAL_SURFACE ( 'NONE', #17231, 0.09999999999999982514, 0.003490658503988666988 ) ;
#523=AXIS2_PLACEMENT_3D ( 'NONE', #65391, #34012, #73934 ) ;
#524=DIRECTION ( 'NONE',  ( 0.000000000000000000, 0.000000000000000000, -1.000000000000000000 ) ) ;
#525=EDGE_LOOP ( 'NONE', ( #12117, #1575, #54740, #85468 ) ) ;
#526=EDGE_LOOP ( 'NONE', ( #35854, #44819 ) ) ;
#527=VERTEX_POINT ( 'NONE', #76672 ) ;
#528=CARTESIAN_POINT ( 'NONE',  ( -3.550000000000028244, 2.500000000000000000, -1.818653347947326138 ) ) ;
#529=AXIS2_PLACEMENT_3D ( 'NONE', #111892, #21574, #91601 ) ;
#530=EDGE_LOOP ( 'NONE', ( #10589, #38123, #90498, #108405 ) ) ;
#531=CARTESIAN_POINT ( 'NONE',  ( -7.950000000000012612, 2.500000000000000000, -2.165063509461101710 ) ) ;
#532=CARTESIAN_POINT ( 'NONE',  ( 5.649999999999934630, 12.50000000000000000, -1.753560074763288457 ) ) ;
#533=CIRCLE ( 'NONE', #113419, 0.06509327318403745899 ) ;
#534=DIRECTION ( 'NONE',  ( 0.000000000000000000, 1.000000000000000000, 0.000000000000000000 ) ) ;
#535=CARTESIAN_POINT ( 'NONE',  ( 0.6499999999999561684, 2.500000000000000000, 1.718653347947321386 ) ) ;
#536=DIRECTION ( 'NONE',  ( -4.274815082592931898E-19, -0.9999939076577903929, -0.003490651415223739937 ) ) ;
#537=DIRECTION ( 'NONE',  ( -0.000000000000000000, 1.000000000000000000, -0.000000000000000000 ) ) ;
#538=CARTESIAN_POINT ( 'NONE',  ( -9.600000000000008527, 2.500000000000000000, 4.230127018922196669 ) ) ;
#540=ORIENTED_EDGE ( 'NONE', *, *, #107770, .T. ) ;
#541=EDGE_CURVE ( 'NONE', #80023, #53300, #26922, .T. ) ;
#542=LINE ( 'NONE', #78496, #27793 ) ;
#543=DIRECTION ( 'NONE',  ( 0.000000000000000000, 0.000000000000000000, 1.000000000000000000 ) ) ;
#544=EDGE_CURVE ( 'NONE', #16388, #101658, #70695, .T. ) ;
#545=ORIENTED_EDGE ( 'NONE', *, *, #127066, .T. ) ;
#546=EDGE_LOOP ( 'NONE', ( #77383, #87063, #10085, #77863 ) ) ;
#547=AXIS2_PLACEMENT_3D ( 'NONE', #38764, #76725, #29556 ) ;
#550=CARTESIAN_POINT ( 'NONE',  ( 1.649999999999951061, 2.500000000000000000, -6.595190528383302109 ) ) ;
#551=EDGE_CURVE ( 'NONE', #109098, #46879, #47726, .T. ) ;
#552=CARTESIAN_POINT ( 'NONE',  ( -7.100000000000017408, 12.50000000000000000, -3.572213422710612374 ) ) ;
#553=CARTESIAN_POINT ( 'NONE',  ( 3.549999999999941203, 2.500000000000000000, 6.048780366869521252 ) ) ;
#554=VECTOR ( 'NONE', #28502, 1000.000000000000000 ) ;
#555=CARTESIAN_POINT ( 'NONE',  ( 8.349999999999923261, 2.500000000000000000, 2.265063509461097357 ) ) ;
#556=DIRECTION ( 'NONE',  ( 0.000000000000000000, 1.000000000000000000, 0.000000000000000000 ) ) ;
#557=AXIS2_PLACEMENT_3D ( 'NONE', #16943, #117096, #120184 ) ;
#558=DIRECTION ( 'NONE',  ( 0.000000000000000000, -0.9999939076577903929, 0.003490651415223739937 ) ) ;
#559=ORIENTED_EDGE ( 'NONE', *, *, #67369, .F. ) ;
#560=ORIENTED_EDGE ( 'NONE', *, *, #7625, .F. ) ;
#561=CONICAL_SURFACE ( 'NONE', #117524, 0.1000000000000002554, 0.003490658503988666988 ) ;
#562=AXIS2_PLACEMENT_3D ( 'NONE', #123402, #33740, #23937 ) ;
#563=ORIENTED_EDGE ( 'NONE', *, *, #110440, .T. ) ;
#564=CONICAL_SURFACE ( 'NONE', #107172, 0.1000000000000002554, 0.003490658503988666988 ) ;
#565=CIRCLE ( 'NONE', #115578, 0.1000000000000002554 ) ;
#566=CIRCLE ( 'NONE', #103280, 0.1000000000000002554 ) ;
#567=ORIENTED_EDGE ( 'NONE', *, *, #110310, .T. ) ;
#568=ORIENTED_EDGE ( 'NONE', *, *, #26797, .F. ) ;
#569=DIRECTION ( 'NONE',  ( -0.000000000000000000, -1.000000000000000000, -0.000000000000000000 ) ) ;
#570=PLANE ( 'NONE',  #77163 ) ;
#571=VECTOR ( 'NONE', #102481, 1000.000000000000000 ) ;
#572=EDGE_LOOP ( 'NONE', ( #97489, #4579, #90813, #4596 ) ) ;
#573=CARTESIAN_POINT ( 'NONE',  ( -12.29999999999999538, 2.500000000000000000, -0.2464101615137742063 ) ) ;
#574=CARTESIAN_POINT ( 'NONE',  ( -13.74999999999998934, 2.500000000000000000, -1.372243186433547812 ) ) ;
#575=DIRECTION ( 'NONE',  ( -0.000000000000000000, -1.000000000000000000, -0.000000000000000000 ) ) ;
#576=DIRECTION ( 'NONE',  ( -4.274815082592931898E-19, -0.9999939076577903929, -0.003490651415223739937 ) ) ;
#577=ORIENTED_EDGE ( 'NONE', *, *, #61831, .F. ) ;
#578=DIRECTION ( 'NONE',  ( 0.000000000000000000, -0.9999939076577903929, 0.003490651415223739937 ) ) ;
#579=AXIS2_PLACEMENT_3D ( 'NONE', #38296, #98473, #105739 ) ;
#580=FACE_OUTER_BOUND ( 'NONE', #16545, .T. ) ;
#581=EDGE_CURVE ( 'NONE', #39745, #108669, #22276, .T. ) ;
#582=ORIENTED_EDGE ( 'NONE', *, *, #51786, .F. ) ;
#583=ORIENTED_EDGE ( 'NONE', *, *, #90235, .F. ) ;
#584=EDGE_LOOP ( 'NONE', ( #71109, #123158, #88532, #32934 ) ) ;
#585=VERTEX_POINT ( 'NONE', #121096 ) ;
#586=DIRECTION ( 'NONE',  ( 0.000000000000000000, 0.000000000000000000, 1.000000000000000000 ) ) ;
#587=DIRECTION ( 'NONE',  ( 0.000000000000000000, 0.000000000000000000, 1.000000000000000000 ) ) ;
#588=CONICAL_SURFACE ( 'NONE', #11049, 0.1000000000000000472, 0.003490658503988666988 ) ;
#589=CARTESIAN_POINT ( 'NONE',  ( -5.200000000000020606, 12.50000000000000000, 3.918623584224383727 ) ) ;
#590=AXIS2_PLACEMENT_3D ( 'NONE', #80178, #48142, #48793 ) ;
#591=AXIS2_PLACEMENT_3D ( 'NONE', #92415, #42040, #13849 ) ;
#592=LINE ( 'NONE', #80479, #106664 ) ;
#593=ADVANCED_FACE ( 'NONE', ( #82479 ), #81179, .T. ) ;
#594=VERTEX_POINT ( 'NONE', #32094 ) ;
#595=CARTESIAN_POINT ( 'NONE',  ( -9.150000000000009237, 12.50000000000000000, -7.253104124594885960 ) ) ;
#596=CARTESIAN_POINT ( 'NONE',  ( 3.299999999999944755, 2.500000000000000000, -2.385244779468109755E-15 ) ) ;
#597=CARTESIAN_POINT ( 'NONE',  ( -5.200000000000024158, 2.500000000000000000, -4.676537180435977881 ) ) ;
#599=EDGE_CURVE ( 'NONE', #33748, #24092, #120865, .T. ) ;
#600=AXIS2_PLACEMENT_3D ( 'NONE', #87066, #7861, #117807 ) ;
#602=AXIS2_PLACEMENT_3D ( 'NONE', #96287, #75361, #105484 ) ;
#604=CARTESIAN_POINT ( 'NONE',  ( 1.249999999999950262, 2.500000000000000000, 7.188010851410848723 ) ) ;
#605=AXIS2_PLACEMENT_3D ( 'NONE', #47938, #87833, #127770 ) ;
#606=EDGE_LOOP ( 'NONE', ( #3129, #48280, #81066, #21095 ) ) ;
#607=ORIENTED_EDGE ( 'NONE', *, *, #84163, .F. ) ;
#608=DIRECTION ( 'NONE',  ( 0.000000000000000000, -0.9999939076577903929, 0.003490651415223739937 ) ) ;
#609=ADVANCED_FACE ( 'NONE', ( #72012 ), #41486, .T. ) ;
#610=DIRECTION ( 'NONE',  ( -0.000000000000000000, -1.000000000000000000, -0.000000000000000000 ) ) ;
#611=FACE_BOUND ( 'NONE', #8184, .T. ) ;
#612=PLANE ( 'NONE',  #122458 ) ;
#613=CIRCLE ( 'NONE', #32042, 0.1000000000000002554 ) ;
#614=DIRECTION ( 'NONE',  ( 0.000000000000000000, 0.000000000000000000, -1.000000000000000000 ) ) ;
#615=CARTESIAN_POINT ( 'NONE',  ( 3.749999999999940492, 12.50000000000000000, 2.857883832488649301 ) ) ;
#616=CIRCLE ( 'NONE', #6853, 0.1000000000000002554 ) ;
#617=AXIS2_PLACEMENT_3D ( 'NONE', #75891, #115817, #26158 ) ;
#618=CIRCLE ( 'NONE', #50816, 0.09999999999999999167 ) ;
#619=DIRECTION ( 'NONE',  ( 0.000000000000000000, 1.000000000000000000, 0.000000000000000000 ) ) ;
#621=CARTESIAN_POINT ( 'NONE',  ( -5.200000000000020606, 12.50000000000000000, 4.048810130592458201 ) ) ;
#622=AXIS2_PLACEMENT_3D ( 'NONE', #18184, #128829, #30615 ) ;
#623=DIRECTION ( 'NONE',  ( 0.000000000000000000, 0.000000000000000000, 1.000000000000000000 ) ) ;
#624=EDGE_LOOP ( 'NONE', ( #73642, #85487, #52293, #4197 ) ) ;
#625=DIRECTION ( 'NONE',  ( -0.000000000000000000, 1.000000000000000000, -0.000000000000000000 ) ) ;
#626=CARTESIAN_POINT ( 'NONE',  ( -2.900000000000029221, 2.500000000000000000, -4.330127018922201643 ) ) ;
#627=AXIS2_PLACEMENT_3D ( 'NONE', #127527, #86948, #126885 ) ;
#628=ORIENTED_EDGE ( 'NONE', *, *, #14488, .T. ) ;
#629=ORIENTED_EDGE ( 'NONE', *, *, #82184, .F. ) ;
#630=CARTESIAN_POINT ( 'NONE',  ( -7.100000000000014744, 2.500000000000000000, 4.330127018922196314 ) ) ;
#631=DIRECTION ( 'NONE',  ( 0.000000000000000000, 0.000000000000000000, 1.000000000000000000 ) ) ;
#632=FACE_BOUND ( 'NONE', #122788, .T. ) ;
#633=CARTESIAN_POINT ( 'NONE',  ( 4.549999999999939426, 12.50000000000000000, -6.430097255199264339 ) ) ;
#634=EDGE_CURVE ( 'NONE', #85204, #14536, #31021, .T. ) ;
#635=CARTESIAN_POINT ( 'NONE',  ( -4.350000000000023626, 2.500000000000000000, 1.818653347947321475 ) ) ;
#636=ORIENTED_EDGE ( 'NONE', *, *, #72588, .T. ) ;
#638=CIRCLE ( 'NONE', #100889, 0.06509327318403745899 ) ;
#639=EDGE_CURVE ( 'NONE', #69112, #15707, #102108, .T. ) ;
#640=FACE_OUTER_BOUND ( 'NONE', #19508, .T. ) ;
#641=ADVANCED_FACE ( 'NONE', ( #70070 ), #118814, .T. ) ;
#642=ORIENTED_EDGE ( 'NONE', *, *, #2599, .T. ) ;
#643=PLANE ( 'NONE',  #15595 ) ;
#645=CIRCLE ( 'NONE', #119784, 0.06509327318403745899 ) ;
#646=EDGE_CURVE ( 'NONE', #35702, #96407, #102093, .T. ) ;
#647=CIRCLE ( 'NONE', #82144, 0.1000000000000002554 ) ;
#648=EDGE_CURVE ( 'NONE', #68126, #33200, #14251, .T. ) ;
#649=CARTESIAN_POINT ( 'NONE',  ( -9.150000000000009237, 12.50000000000000000, -7.122917578226811486 ) ) ;
#650=EDGE_CURVE ( 'NONE', #29270, #9679, #104147, .T. ) ;
#651=CARTESIAN_POINT ( 'NONE',  ( 12.69999999999989804, 12.50000000000000000, 0.3464101615137735735 ) ) ;
#652=AXIS2_PLACEMENT_3D ( 'NONE', #68658, #36645, #49043 ) ;
#653=VECTOR ( 'NONE', #20079, 1000.000000000000000 ) ;
#654=ORIENTED_EDGE ( 'NONE', *, *, #100999, .T. ) ;
#655=AXIS2_PLACEMENT_3D ( 'NONE', #129245, #87973, #78193 ) ;
#656=CARTESIAN_POINT ( 'NONE',  ( -12.69999999999999218, 2.500000000000000000, -4.676537180435975216 ) ) ;
#657=ADVANCED_FACE ( 'NONE', ( #109342 ), #64432, .T. ) ;
#658=DIRECTION ( 'NONE',  ( 0.000000000000000000, 0.000000000000000000, 1.000000000000000000 ) ) ;
#659=PLANE ( 'NONE',  #63936 ) ;
#660=AXIS2_PLACEMENT_3D ( 'NONE', #121579, #43705, #10965 ) ;
#661=AXIS2_PLACEMENT_3D ( 'NONE', #47904, #18431, #106796 ) ;
#662=ORIENTED_EDGE ( 'NONE', *, *, #127719, .F. ) ;
#663=EDGE_LOOP ( 'NONE', ( #88729, #95449 ) ) ;
#664=DIRECTION ( 'NONE',  ( -0.000000000000000000, 1.000000000000000000, -0.000000000000000000 ) ) ;
#665=ADVANCED_FACE ( 'NONE', ( #41271 ), #71337, .T. ) ;
#666=CONICAL_SURFACE ( 'NONE', #11119, 0.1000000000000002554, 0.003490658503988666988 ) ;
#667=ORIENTED_EDGE ( 'NONE', *, *, #63347, .F. ) ;
#668=DIRECTION ( 'NONE',  ( 0.000000000000000000, 0.000000000000000000, -1.000000000000000000 ) ) ;
#669=FACE_OUTER_BOUND ( 'NONE', #29516, .T. ) ;
#670=LINE ( 'NONE', #50417, #27795 ) ;
#671=ORIENTED_EDGE ( 'NONE', *, *, #14169, .F. ) ;
#672=DIRECTION ( 'NONE',  ( 0.000000000000000000, -0.9999939076577903929, 0.003490651415223739937 ) ) ;
#673=CARTESIAN_POINT ( 'NONE',  ( 10.84999999999991260, 2.500000000000000000, -2.165063509461101710 ) ) ;
#674=DIRECTION ( 'NONE',  ( 0.000000000000000000, 0.000000000000000000, 1.000000000000000000 ) ) ;
#675=PLANE ( 'NONE',  #37128 ) ;
#676=CARTESIAN_POINT ( 'NONE',  ( 11.89999999999990798, 12.50000000000000000, 4.676537180435972552 ) ) ;
#677=DIRECTION ( 'NONE',  ( 0.000000000000000000, 1.000000000000000000, 0.000000000000000000 ) ) ;
#678=CIRCLE ( 'NONE', #52921, 0.09999999999999982514 ) ;
#679=EDGE_LOOP ( 'NONE', ( #46494, #123936 ) ) ;
#680=EDGE_LOOP ( 'NONE', ( #77072, #102505 ) ) ;
#681=FACE_OUTER_BOUND ( 'NONE', #89916, .T. ) ;
#682=EDGE_LOOP ( 'NONE', ( #37408, #91161 ) ) ;
#683=DIRECTION ( 'NONE',  ( -0.000000000000000000, -1.000000000000000000, -0.000000000000000000 ) ) ;
#684=ORIENTED_EDGE ( 'NONE', *, *, #99808, .F. ) ;
#685=ORIENTED_EDGE ( 'NONE', *, *, #2709, .T. ) ;
#686=EDGE_LOOP ( 'NONE', ( #115705, #18829, #20205, #100093, #70594, #129048 ) ) ;
#687=PLANE ( 'NONE',  #43815 ) ;
#688=AXIS2_PLACEMENT_3D ( 'NONE', #1248, #41199, #81111 ) ;
#689=AXIS2_PLACEMENT_3D ( 'NONE', #46058, #103692, #13992 ) ;
#690=DIRECTION ( 'NONE',  ( 0.000000000000000000, -0.9999939076577903929, 0.003490651415223739937 ) ) ;
#691=AXIS2_PLACEMENT_3D ( 'NONE', #109981, #91413, #73068 ) ;
#692=DIRECTION ( 'NONE',  ( 0.000000000000000000, 1.000000000000000000, 0.000000000000000000 ) ) ;
#693=DIRECTION ( 'NONE',  ( 0.000000000000000000, 0.000000000000000000, 1.000000000000000000 ) ) ;
#694=DIRECTION ( 'NONE',  ( 0.000000000000000000, 0.000000000000000000, 1.000000000000000000 ) ) ;
#696=CARTESIAN_POINT ( 'NONE',  ( -0.4000000000000404898, 2.500000000000000000, 5.022947341949748790 ) ) ;
#697=DIRECTION ( 'NONE',  ( -0.000000000000000000, -1.000000000000000000, -0.000000000000000000 ) ) ;
#698=CIRCLE ( 'NONE', #115711, 0.1000000000000002554 ) ;
#699=CONICAL_SURFACE ( 'NONE', #23694, 0.1000000000000002554, 0.003490658503988666988 ) ;
#700=PLANE ( 'NONE',  #114607 ) ;
#701=CIRCLE ( 'NONE', #124037, 0.06509327318403745899 ) ;
#702=VERTEX_POINT ( 'NONE', #42561 ) ;
#703=AXIS2_PLACEMENT_3D ( 'NONE', #90090, #21364, #80944 ) ;
#704=EDGE_CURVE ( 'NONE', #22628, #35194, #74910, .T. ) ;
#705=FACE_OUTER_BOUND ( 'NONE', #8845, .T. ) ;
#706=ORIENTED_EDGE ( 'NONE', *, *, #56081, .F. ) ;
#707=EDGE_LOOP ( 'NONE', ( #52225, #86557 ) ) ;
#708=CARTESIAN_POINT ( 'NONE',  ( -9.350000000000004974, 2.500000000000000000, 6.841600689897072485 ) ) ;
#709=AXIS2_PLACEMENT_3D ( 'NONE', #109330, #19668, #66810 ) ;
#710=PLANE ( 'NONE',  #109123 ) ;
#711=ADVANCED_FACE ( 'NONE', ( #60886 ), #91621, .T. ) ;
#713=CARTESIAN_POINT ( 'NONE',  ( 4.549999999999939426, 12.50000000000000000, -2.230156782645139391 ) ) ;
#714=AXIS2_PLACEMENT_3D ( 'NONE', #88680, #120083, #118780 ) ;
#715=DIRECTION ( 'NONE',  ( 0.000000000000000000, 1.000000000000000000, 0.000000000000000000 ) ) ;
#716=CIRCLE ( 'NONE', #2872, 0.06509327318403745899 ) ;
#717=CARTESIAN_POINT ( 'NONE',  ( -13.94999999999998685, 2.500000000000000000, 1.918653347947325338 ) ) ;
#718=ORIENTED_EDGE ( 'NONE', *, *, #25746, .T. ) ;
#719=AXIS2_PLACEMENT_3D ( 'NONE', #63117, #13369, #50723 ) ;
#720=ORIENTED_EDGE ( 'NONE', *, *, #108181, .T. ) ;
#721=CARTESIAN_POINT ( 'NONE',  ( 3.349999999999945466, 2.500000000000000000, -7.188010851410854052 ) ) ;
#722=ORIENTED_EDGE ( 'NONE', *, *, #47754, .T. ) ;
#723=DIRECTION ( 'NONE',  ( -0.000000000000000000, -1.000000000000000000, -0.000000000000000000 ) ) ;
#724=ORIENTED_EDGE ( 'NONE', *, *, #22817, .T. ) ;
#725=ORIENTED_EDGE ( 'NONE', *, *, #32189, .T. ) ;
#726=FACE_OUTER_BOUND ( 'NONE', #107954, .T. ) ;
#727=CARTESIAN_POINT ( 'NONE',  ( 21.23528140090950700, -2.699413673072311948, -2.293764360948876480 ) ) ;
#728=CARTESIAN_POINT ( 'NONE',  ( 11.04999999999991012, 12.50000000000000000, -1.753560074763288679 ) ) ;
#729=DIRECTION ( 'NONE',  ( 0.000000000000000000, 1.000000000000000000, 0.000000000000000000 ) ) ;
#730=CARTESIAN_POINT ( 'NONE',  ( 17.50000000000000000, 2.083333333333332593, 4.000000000000000000 ) ) ;
#731=ORIENTED_EDGE ( 'NONE', *, *, #47779, .F. ) ;
#732=DIRECTION ( 'NONE',  ( 0.000000000000000000, -0.9999939076577903929, 0.003490651415223739937 ) ) ;
#733=DIRECTION ( 'NONE',  ( 0.000000000000000000, -0.9999939076577903929, 0.003490651415223739937 ) ) ;
#734=AXIS2_PLACEMENT_3D ( 'NONE', #117084, #126934, #27414 ) ;
#735=AXIS2_PLACEMENT_3D ( 'NONE', #18059, #116896, #17403 ) ;
#736=DIRECTION ( 'NONE',  ( 0.000000000000000000, 0.000000000000000000, 1.000000000000000000 ) ) ;
#737=LINE ( 'NONE', #40701, #109967 ) ;
#738=DIRECTION ( 'NONE',  ( 0.000000000000000000, -0.9999939076577903929, 0.003490651415223739937 ) ) ;
#739=EDGE_CURVE ( 'NONE', #98477, #23899, #10067, .T. ) ;
#740=VERTEX_POINT ( 'NONE', #49801 ) ;
#741=CONICAL_SURFACE ( 'NONE', #119881, 0.1000000000000002554, 0.003490658503988666988 ) ;
#742=ORIENTED_EDGE ( 'NONE', *, *, #43010, .F. ) ;
#743=AXIS2_PLACEMENT_3D ( 'NONE', #53506, #3744, #21453 ) ;
#744=VECTOR ( 'NONE', #21845, 1000.000000000000000 ) ;
#745=CARTESIAN_POINT ( 'NONE',  ( 12.29999999999990656, 2.500000000000000000, 4.083716857408421497 ) ) ;
#747=CARTESIAN_POINT ( 'NONE',  ( 1.049999999999952971, 2.500000000000000000, 6.148780366869520897 ) ) ;
#748=DIRECTION ( 'NONE',  ( 0.000000000000000000, 0.000000000000000000, 1.000000000000000000 ) ) ;
#749=EDGE_CURVE ( 'NONE', #15903, #100174, #108344, .T. ) ;
#750=CIRCLE ( 'NONE', #90638, 0.09999999999999982514 ) ;
#751=CONICAL_SURFACE ( 'NONE', #73913, 0.09999999999999999167, 0.003490658503988666988 ) ;
#752=CIRCLE ( 'NONE', #82443, 0.09999999999999982514 ) ;
#753=AXIS2_PLACEMENT_3D ( 'NONE', #109386, #92317, #2000 ) ;
#754=ADVANCED_FACE ( 'NONE', ( #62828 ), #122939, .T. ) ;
#755=EDGE_LOOP ( 'NONE', ( #13923, #69922 ) ) ;
#756=DIRECTION ( 'NONE',  ( -0.000000000000000000, 1.000000000000000000, -0.000000000000000000 ) ) ;
#757=FACE_OUTER_BOUND ( 'NONE', #96203, .T. ) ;
#758=FACE_OUTER_BOUND ( 'NONE', #31325, .T. ) ;
#759=ADVANCED_FACE ( 'NONE', ( #5814 ), #45670, .T. ) ;
#760=DIRECTION ( 'NONE',  ( 0.000000000000000000, 0.000000000000000000, 1.000000000000000000 ) ) ;
#761=FACE_OUTER_BOUND ( 'NONE', #38545, .T. ) ;
#762=EDGE_CURVE ( 'NONE', #24428, #9737, #115114, .T. ) ;
#763=ORIENTED_EDGE ( 'NONE', *, *, #42656, .T. ) ;
#764=EDGE_CURVE ( 'NONE', #127196, #103587, #43532, .T. ) ;
#765=CARTESIAN_POINT ( 'NONE',  ( -1.650000000000034772, 2.500000000000000000, 6.395190528383296602 ) ) ;
#766=FACE_OUTER_BOUND ( 'NONE', #35567, .T. ) ;
#767=CARTESIAN_POINT ( 'NONE',  ( -13.09999999999999254, 2.500000000000000000, -4.083716857408424161 ) ) ;
#768=AXIS2_PLACEMENT_3D ( 'NONE', #63578, #93039, #112031 ) ;
#769=CARTESIAN_POINT ( 'NONE',  ( -4.550000000000022915, 12.50000000000000000, 6.430097255199259010 ) ) ;
#770=EDGE_LOOP ( 'NONE', ( #91474, #18313 ) ) ;
#771=EDGE_LOOP ( 'NONE', ( #4054, #86586, #92861, #126394 ) ) ;
#772=FACE_OUTER_BOUND ( 'NONE', #113605, .T. ) ;
#773=CARTESIAN_POINT ( 'NONE',  ( -1.250000000000001110, 12.50000000000000000, -2.230156782645139391 ) ) ;
#774=LINE ( 'NONE', #119915, #1580 ) ;
#775=AXIS2_PLACEMENT_3D ( 'NONE', #126173, #107164, #7020 ) ;
#777=VECTOR ( 'NONE', #12550, 1000.000000000000000 ) ;
#778=CIRCLE ( 'NONE', #90671, 0.1000000000000002554 ) ;
#779=DIRECTION ( 'NONE',  ( -0.000000000000000000, 1.000000000000000000, -0.000000000000000000 ) ) ;
#780=CARTESIAN_POINT ( 'NONE',  ( 4.999999999999938716, 2.500000000000000000, -5.022947341949754119 ) ) ;
#781=VERTEX_POINT ( 'NONE', #43204 ) ;
#782=CARTESIAN_POINT ( 'NONE',  ( -9.150000000000009237, 12.50000000000000000, -1.407149913249512663 ) ) ;
#783=VECTOR ( 'NONE', #10300, 1000.000000000000000 ) ;
#784=ORIENTED_EDGE ( 'NONE', *, *, #22311, .F. ) ;
#786=CARTESIAN_POINT ( 'NONE',  ( 8.099999999999923261, 2.500000000000000000, -4.676537180435978769 ) ) ;
#787=VECTOR ( 'NONE', #9613, 1000.000000000000000 ) ;
#788=ADVANCED_FACE ( 'NONE', ( #54924 ), #83121, .T. ) ;
#789=ORIENTED_EDGE ( 'NONE', *, *, #47381, .F. ) ;
#791=CARTESIAN_POINT ( 'NONE',  ( 3.677964504776914723, 2.499999999999999112, -8.999999999999996447 ) ) ;
#792=ORIENTED_EDGE ( 'NONE', *, *, #103180, .T. ) ;
#793=ORIENTED_EDGE ( 'NONE', *, *, #120546, .F. ) ;
#794=EDGE_CURVE ( 'NONE', #29548, #67957, #37265, .T. ) ;
#795=VECTOR ( 'NONE', #27229, 1000.000000000000000 ) ;
#796=CARTESIAN_POINT ( 'NONE',  ( 3.949999999999938005, 2.500000000000000000, 6.841600689897072485 ) ) ;
#798=ORIENTED_EDGE ( 'NONE', *, *, #111103, .F. ) ;
#799=EDGE_CURVE ( 'NONE', #50587, #11702, #35310, .T. ) ;
#801=CARTESIAN_POINT ( 'NONE',  ( 10.64999999999990976, 2.500000000000000000, -6.841600689897077814 ) ) ;
#802=CIRCLE ( 'NONE', #73974, 0.06509327318403745899 ) ;
#803=DIRECTION ( 'NONE',  ( 0.000000000000000000, 0.000000000000000000, 1.000000000000000000 ) ) ;
#804=CONICAL_SURFACE ( 'NONE', #21660, 0.1000000000000000472, 0.003490658503988666988 ) ;
#806=CARTESIAN_POINT ( 'NONE',  ( -12.09999999999999609, 12.50000000000000000, -0.6928203230275501445 ) ) ;
#807=EDGE_CURVE ( 'NONE', #38593, #8229, #116661, .T. ) ;
#808=CARTESIAN_POINT ( 'NONE',  ( 7.899999999999924860, 2.500000000000000000, 4.330127018922196314 ) ) ;
#809=AXIS2_PLACEMENT_3D ( 'NONE', #65694, #5470, #6118 ) ;
#810=FACE_OUTER_BOUND ( 'NONE', #5290, .T. ) ;
#811=EDGE_CURVE ( 'NONE', #122569, #115231, #52448, .T. ) ;
#812=EDGE_CURVE ( 'NONE', #65686, #2207, #23202, .T. ) ;
#813=CIRCLE ( 'NONE', #90706, 0.1000000000000002554 ) ;
#814=ORIENTED_EDGE ( 'NONE', *, *, #96816, .F. ) ;
#815=ORIENTED_EDGE ( 'NONE', *, *, #44054, .T. ) ;
#816=EDGE_CURVE ( 'NONE', #96927, #17385, #73280, .T. ) ;
#817=ORIENTED_EDGE ( 'NONE', *, *, #54697, .T. ) ;
#818=DIRECTION ( 'NONE',  ( 0.000000000000000000, 0.000000000000000000, 1.000000000000000000 ) ) ;
#819=PLANE ( 'NONE',  #11518 ) ;
#820=DIRECTION ( 'NONE',  ( 0.000000000000000000, 1.000000000000000000, 0.000000000000000000 ) ) ;
#821=ORIENTED_EDGE ( 'NONE', *, *, #89628, .T. ) ;
#822=ORIENTED_EDGE ( 'NONE', *, *, #76466, .F. ) ;
#823=FACE_BOUND ( 'NONE', #115451, .T. ) ;
#824=ORIENTED_EDGE ( 'NONE', *, *, #54300, .F. ) ;
#825=DIRECTION ( 'NONE',  ( -0.000000000000000000, 1.000000000000000000, -0.000000000000000000 ) ) ;
#826=DIRECTION ( 'NONE',  ( 0.000000000000000000, 0.000000000000000000, -1.000000000000000000 ) ) ;
#827=EDGE_CURVE ( 'NONE', #45964, #73617, #113863, .T. ) ;
#828=CARTESIAN_POINT ( 'NONE',  ( -7.500000000000015099, 12.50000000000000000, -5.022947341949754119 ) ) ;
#829=DIRECTION ( 'NONE',  ( 0.000000000000000000, 0.000000000000000000, 1.000000000000000000 ) ) ;
#831=CARTESIAN_POINT ( 'NONE',  ( 6.849999999999929479, 2.500000000000000000, 6.841600689897072485 ) ) ;
#832=DIRECTION ( 'NONE',  ( -0.000000000000000000, 1.000000000000000000, -0.000000000000000000 ) ) ;
#833=FACE_OUTER_BOUND ( 'NONE', #13489, .T. ) ;
#834=CARTESIAN_POINT ( 'NONE',  ( 11.44999999999990870, 2.500000000000000000, 6.741600689897071952 ) ) ;
#835=AXIS2_PLACEMENT_3D ( 'NONE', #53529, #43086, #101340 ) ;
#836=CIRCLE ( 'NONE', #2896, 0.06509327318403745899 ) ;
#837=CARTESIAN_POINT ( 'NONE',  ( -10.85000000000000142, 2.500000000000000000, 6.495190528383297135 ) ) ;
#838=CARTESIAN_POINT ( 'NONE',  ( 0.8499999999999557909, 2.500000000000000000, -7.088010851410853519 ) ) ;
#839=CIRCLE ( 'NONE', #38428, 0.1000000000000002554 ) ;
#840=EDGE_LOOP ( 'NONE', ( #98615, #3304 ) ) ;
#841=EDGE_LOOP ( 'NONE', ( #59112, #57960 ) ) ;
#842=ORIENTED_EDGE ( 'NONE', *, *, #93315, .F. ) ;
#843=AXIS2_PLACEMENT_3D ( 'NONE', #119388, #6837, #18621 ) ;
#844=VERTEX_POINT ( 'NONE', #113198 ) ;
#845=DIRECTION ( 'NONE',  ( 0.000000000000000000, -0.9999939076577903929, 0.003490651415223739937 ) ) ;
#846=CIRCLE ( 'NONE', #74008, 0.1000000000000002554 ) ;
#847=DIRECTION ( 'NONE',  ( 0.000000000000000000, -0.000000000000000000, 1.000000000000000000 ) ) ;
#848=EDGE_LOOP ( 'NONE', ( #80324, #87937, #52019, #60747 ) ) ;
#849=ORIENTED_EDGE ( 'NONE', *, *, #54920, .F. ) ;
#850=VERTEX_POINT ( 'NONE', #54290 ) ;
#851=DIRECTION ( 'NONE',  ( 0.000000000000000000, 0.000000000000000000, -1.000000000000000000 ) ) ;
#852=CIRCLE ( 'NONE', #28042, 0.06509327318403745899 ) ;
#853=AXIS2_PLACEMENT_3D ( 'NONE', #56388, #105508, #86495 ) ;
#854=VECTOR ( 'NONE', #29476, 1000.000000000000000 ) ;
#855=DIRECTION ( 'NONE',  ( 0.000000000000000000, 0.000000000000000000, -1.000000000000000000 ) ) ;
#856=CARTESIAN_POINT ( 'NONE',  ( 6.449999999999931788, 2.500000000000000000, -2.411473670974877859 ) ) ;
#857=LINE ( 'NONE', #20508, #66802 ) ;
#858=DIRECTION ( 'NONE',  ( -0.000000000000000000, 1.000000000000000000, -0.000000000000000000 ) ) ;
#859=DIRECTION ( 'NONE',  ( 0.000000000000000000, 0.000000000000000000, -1.000000000000000000 ) ) ;
#860=AXIS2_PLACEMENT_3D ( 'NONE', #49692, #9095, #71903 ) ;
#861=CARTESIAN_POINT ( 'NONE',  ( -6.650000000000014566, 2.500000000000000000, 1.372243186433545370 ) ) ;
#862=EDGE_CURVE ( 'NONE', #68242, #18421, #106821, .T. ) ;
#863=ORIENTED_EDGE ( 'NONE', *, *, #58832, .F. ) ;
#864=FACE_OUTER_BOUND ( 'NONE', #76237, .T. ) ;
#865=ORIENTED_EDGE ( 'NONE', *, *, #82965, .F. ) ;
#866=ORIENTED_EDGE ( 'NONE', *, *, #8700, .T. ) ;
#867=EDGE_CURVE ( 'NONE', #70717, #56812, #94301, .T. ) ;
#868=VERTEX_POINT ( 'NONE', #103399 ) ;
#869=CONICAL_SURFACE ( 'NONE', #90748, 0.1000000000000002554, 0.003490658503988666988 ) ;
#870=FACE_OUTER_BOUND ( 'NONE', #102181, .T. ) ;
#872=ORIENTED_EDGE ( 'NONE', *, *, #43821, .T. ) ;
#873=EDGE_LOOP ( 'NONE', ( #111150, #114806, #127248, #113031 ) ) ;
#874=ORIENTED_EDGE ( 'NONE', *, *, #56407, .T. ) ;
#875=AXIS2_PLACEMENT_3D ( 'NONE', #27933, #16153, #45657 ) ;
#876=CARTESIAN_POINT ( 'NONE',  ( 4.349999999999940137, 2.500000000000000000, -6.741600689897078169 ) ) ;
#877=EDGE_CURVE ( 'NONE', #50948, #78678, #39949, .T. ) ;
#878=DIRECTION ( 'NONE',  ( -0.000000000000000000, -1.000000000000000000, -0.000000000000000000 ) ) ;
#879=DIRECTION ( 'NONE',  ( -4.274815082592931898E-19, -0.9999939076577903929, -0.003490651415223739937 ) ) ;
#880=CARTESIAN_POINT ( 'NONE',  ( 12.49999999999993960, 2.500000000000000000, -4.330127018922201643 ) ) ;
#882=DIRECTION ( 'NONE',  ( 0.000000000000000000, 0.000000000000000000, 1.000000000000000000 ) ) ;
#883=DIRECTION ( 'NONE',  ( 0.000000000000000000, 0.000000000000000000, -1.000000000000000000 ) ) ;
#884=CIRCLE ( 'NONE', #4973, 0.09999999999999982514 ) ;
#885=VERTEX_POINT ( 'NONE', #22909 ) ;
#886=CARTESIAN_POINT ( 'NONE',  ( -2.100000000000033396, 12.50000000000000000, 0.7579135962115869374 ) ) ;
#887=ORIENTED_EDGE ( 'NONE', *, *, #7825, .F. ) ;
#889=CARTESIAN_POINT ( 'NONE',  ( 6.249999999999930722, 2.500000000000000000, 7.088010851410848190 ) ) ;
#890=VERTEX_POINT ( 'NONE', #3895 ) ;
#891=CARTESIAN_POINT ( 'NONE',  ( 13.29999999999990301, 2.500000000000000000, 4.230127018922196669 ) ) ;
#892=DIRECTION ( 'NONE',  ( 0.000000000000000000, 0.000000000000000000, -1.000000000000000000 ) ) ;
#893=ORIENTED_EDGE ( 'NONE', *, *, #26645, .T. ) ;
#894=AXIS2_PLACEMENT_3D ( 'NONE', #69015, #31684, #11389 ) ;
#895=DIRECTION ( 'NONE',  ( -0.000000000000000000, -1.000000000000000000, -0.000000000000000000 ) ) ;
#896=VERTEX_POINT ( 'NONE', #13049 ) ;
#897=ORIENTED_EDGE ( 'NONE', *, *, #96445, .F. ) ;
#898=DIRECTION ( 'NONE',  ( 0.000000000000000000, 0.000000000000000000, -1.000000000000000000 ) ) ;
#899=CARTESIAN_POINT ( 'NONE',  ( -9.150000000000005684, 12.50000000000000000, 5.737276932171707422 ) ) ;
#900=CARTESIAN_POINT ( 'NONE',  ( -6.850000000000013856, 2.500000000000000000, 2.411473670974873862 ) ) ;
#901=DIRECTION ( 'NONE',  ( 0.000000000000000000, -0.9999939076577903929, 0.003490651415223739937 ) ) ;
#902=CARTESIAN_POINT ( 'NONE',  ( -12.29999999999999361, 2.500000000000000000, 4.083716857408420609 ) ) ;
#903=ORIENTED_EDGE ( 'NONE', *, *, #37923, .T. ) ;
#904=AXIS2_PLACEMENT_3D ( 'NONE', #50770, #39687, #101161 ) ;
#905=CARTESIAN_POINT ( 'NONE',  ( -7.100000000000017408, 2.500000000000000000, -3.537306695894649966 ) ) ;
#906=VECTOR ( 'NONE', #123801, 1000.000000000000000 ) ;
#907=VERTEX_POINT ( 'NONE', #43851 ) ;
#908=AXIS2_PLACEMENT_3D ( 'NONE', #39778, #99970, #59420 ) ;
#909=CARTESIAN_POINT ( 'NONE',  ( -2.300000000000033573, 12.50000000000000000, 0.3464101615137735735 ) ) ;
#910=CARTESIAN_POINT ( 'NONE',  ( -12.89999999999999147, 12.50000000000000000, -4.330127018922198978 ) ) ;
#911=EDGE_CURVE ( 'NONE', #33867, #20692, #45126, .T. ) ;
#913=EDGE_CURVE ( 'NONE', #12403, #70927, #57523, .T. ) ;
#914=DIRECTION ( 'NONE',  ( -0.000000000000000000, -1.000000000000000000, -0.000000000000000000 ) ) ;
#915=DIRECTION ( 'NONE',  ( 0.000000000000000000, 0.000000000000000000, 1.000000000000000000 ) ) ;
#916=CARTESIAN_POINT ( 'NONE',  ( 9.149999999999920419, 12.50000000000000000, -7.188010851410854052 ) ) ;
#918=ADVANCED_FACE ( 'NONE', ( #56211 ), #90091, .T. ) ;
#919=DIRECTION ( 'NONE',  ( -0.000000000000000000, 1.000000000000000000, -0.000000000000000000 ) ) ;
#920=ORIENTED_EDGE ( 'NONE', *, *, #122375, .T. ) ;
#922=AXIS2_PLACEMENT_3D ( 'NONE', #51766, #120500, #81225 ) ;
#923=DIRECTION ( 'NONE',  ( -0.000000000000000000, 1.000000000000000000, -0.000000000000000000 ) ) ;
#924=DIRECTION ( 'NONE',  ( 0.000000000000000000, 0.000000000000000000, 1.000000000000000000 ) ) ;
#925=ADVANCED_FACE ( 'NONE', ( #77779 ), #67090, .T. ) ;
#926=VECTOR ( 'NONE', #84922, 1000.000000000000000 ) ;
#927=EDGE_CURVE ( 'NONE', #8077, #54326, #77574, .T. ) ;
#928=CONICAL_SURFACE ( 'NONE', #59441, 0.1000000000000002554, 0.003490658503988666988 ) ;
#929=CIRCLE ( 'NONE', #99137, 0.1000000000000002554 ) ;
#930=ADVANCED_FACE ( 'NONE', ( #36609 ), #113094, .T. ) ;
#931=EDGE_LOOP ( 'NONE', ( #99662, #13541, #5965, #64093 ) ) ;
#932=CARTESIAN_POINT ( 'NONE',  ( -1.050000000000038680, 2.500000000000000000, 6.841600689897072485 ) ) ;
#933=AXIS2_PLACEMENT_3D ( 'NONE', #28967, #119255, #53600 ) ;
#934=AXIS2_PLACEMENT_3D ( 'NONE', #92141, #51598, #2459 ) ;
#935=VERTEX_POINT ( 'NONE', #86970 ) ;
#936=AXIS2_PLACEMENT_3D ( 'NONE', #25174, #95863, #96481 ) ;
#937=ORIENTED_EDGE ( 'NONE', *, *, #15718, .T. ) ;
#938=CARTESIAN_POINT ( 'NONE',  ( -5.400000000000019895, 2.500000000000000000, -0.1000000000000022815 ) ) ;
#939=ORIENTED_EDGE ( 'NONE', *, *, #27834, .T. ) ;
#940=DIRECTION ( 'NONE',  ( -0.000000000000000000, -1.000000000000000000, -0.000000000000000000 ) ) ;
#941=DIRECTION ( 'NONE',  ( -0.000000000000000000, 1.000000000000000000, -0.000000000000000000 ) ) ;
#942=VERTEX_POINT ( 'NONE', #107897 ) ;
#943=CIRCLE ( 'NONE', #59460, 0.06509327318403745899 ) ;
#944=AXIS2_PLACEMENT_3D ( 'NONE', #66648, #73902, #113841 ) ;
#945=DIRECTION ( 'NONE',  ( 0.000000000000000000, 0.000000000000000000, 1.000000000000000000 ) ) ;
#946=DIRECTION ( 'NONE',  ( 0.000000000000000000, 0.000000000000000000, 1.000000000000000000 ) ) ;
#947=CARTESIAN_POINT ( 'NONE',  ( 6.649999999999930189, 2.500000000000000000, 7.188010851410848723 ) ) ;
#948=VERTEX_POINT ( 'NONE', #118360 ) ;
#949=VERTEX_POINT ( 'NONE', #77156 ) ;
#950=ORIENTED_EDGE ( 'NONE', *, *, #128216, .T. ) ;
#951=FACE_OUTER_BOUND ( 'NONE', #103034, .T. ) ;
#952=FACE_OUTER_BOUND ( 'NONE', #45269, .T. ) ;
#953=FACE_BOUND ( 'NONE', #20794, .T. ) ;
#954=ORIENTED_EDGE ( 'NONE', *, *, #127003, .F. ) ;
#955=DIRECTION ( 'NONE',  ( 0.000000000000000000, 1.000000000000000000, 0.000000000000000000 ) ) ;
#956=LINE ( 'NONE', #120732, #100379 ) ;
#957=AXIS2_PLACEMENT_3D ( 'NONE', #47353, #106264, #5468 ) ;
#958=ORIENTED_EDGE ( 'NONE', *, *, #56440, .F. ) ;
#959=DIRECTION ( 'NONE',  ( -0.000000000000000000, 1.000000000000000000, -0.000000000000000000 ) ) ;
#960=DIRECTION ( 'NONE',  ( -0.000000000000000000, 1.000000000000000000, -0.000000000000000000 ) ) ;
#961=FACE_OUTER_BOUND ( 'NONE', #54640, .T. ) ;
#963=CARTESIAN_POINT ( 'NONE',  ( -12.49999999999999289, 2.500000000000000000, -5.022947341949751454 ) ) ;
#964=CARTESIAN_POINT ( 'NONE',  ( 6.249999999999930722, 2.500000000000000000, -1.472243186433550122 ) ) ;
#965=ADVANCED_FACE ( 'NONE', ( #27385 ), #66674, .T. ) ;
#966=DIRECTION ( 'NONE',  ( -4.274815082592931898E-19, -0.9999939076577903929, -0.003490651415223739937 ) ) ;
#967=DIRECTION ( 'NONE',  ( -0.000000000000000000, 1.000000000000000000, -0.000000000000000000 ) ) ;
#968=EDGE_CURVE ( 'NONE', #31124, #37879, #75433, .T. ) ;
#969=AXIS2_PLACEMENT_3D ( 'NONE', #101280, #111743, #11603 ) ;
#970=AXIS2_PLACEMENT_3D ( 'NONE', #65992, #45725, #47657 ) ;
#971=ORIENTED_EDGE ( 'NONE', *, *, #117601, .T. ) ;
#972=ORIENTED_EDGE ( 'NONE', *, *, #67206, .F. ) ;
#973=EDGE_CURVE ( 'NONE', #55129, #47060, #16904, .T. ) ;
#974=ORIENTED_EDGE ( 'NONE', *, *, #58775, .T. ) ;
#975=ORIENTED_EDGE ( 'NONE', *, *, #76084, .F. ) ;
#976=CARTESIAN_POINT ( 'NONE',  ( -1.650000000000035660, 12.50000000000000000, 7.188010851410848723 ) ) ;
#977=EDGE_CURVE ( 'NONE', #39788, #14289, #44141, .T. ) ;
#978=DIRECTION ( 'NONE',  ( -0.000000000000000000, 1.000000000000000000, -0.000000000000000000 ) ) ;
#979=ORIENTED_EDGE ( 'NONE', *, *, #25487, .F. ) ;
#980=FACE_BOUND ( 'NONE', #85138, .T. ) ;
#981=DIRECTION ( 'NONE',  ( 0.000000000000000000, 0.000000000000000000, 1.000000000000000000 ) ) ;
#982=EDGE_CURVE ( 'NONE', #98740, #31546, #87607, .T. ) ;
#983=AXIS2_PLACEMENT_3D ( 'NONE', #115362, #85915, #18479 ) ;
#984=DIRECTION ( 'NONE',  ( 0.000000000000000000, -0.9999939076577903929, 0.003490651415223739937 ) ) ;
#985=EDGE_CURVE ( 'NONE', #72823, #32164, #4398, .T. ) ;
#986=DIRECTION ( 'NONE',  ( 0.000000000000000000, -0.9999939076577903929, 0.003490651415223739937 ) ) ;
#987=AXIS2_PLACEMENT_3D ( 'NONE', #18990, #69386, #100156 ) ;
#988=CARTESIAN_POINT ( 'NONE',  ( 12.89999999999990266, 2.500000000000000000, -5.022947341949754119 ) ) ;
#989=DIRECTION ( 'NONE',  ( 0.000000000000000000, 1.000000000000000000, 0.000000000000000000 ) ) ;
#990=DIRECTION ( 'NONE',  ( 0.000000000000000000, -0.000000000000000000, 1.000000000000000000 ) ) ;
#991=DIRECTION ( 'NONE',  ( 0.000000000000000000, 0.000000000000000000, 1.000000000000000000 ) ) ;
#992=DIRECTION ( 'NONE',  ( 0.000000000000000000, 0.000000000000000000, 1.000000000000000000 ) ) ;
#994=EDGE_CURVE ( 'NONE', #52844, #31178, #17573, .T. ) ;
#995=ORIENTED_EDGE ( 'NONE', *, *, #125991, .T. ) ;
#996=VECTOR ( 'NONE', #128972, 1000.000000000000000 ) ;
#997=VERTEX_POINT ( 'NONE', #98709 ) ;
#998=EDGE_LOOP ( 'NONE', ( #19854, #122613 ) ) ;
#999=VECTOR ( 'NONE', #84850, 1000.000000000000000 ) ;
#1001=EDGE_LOOP ( 'NONE', ( #92741, #66939, #84110, #76480 ) ) ;
#1002=FACE_OUTER_BOUND ( 'NONE', #2724, .T. ) ;
#1003=AXIS2_PLACEMENT_3D ( 'NONE', #62666, #82305, #12880 ) ;
#1004=VERTEX_POINT ( 'NONE', #49002 ) ;
#1005=CIRCLE ( 'NONE', #90886, 0.09999999999999999167 ) ;
#1006=CARTESIAN_POINT ( 'NONE',  ( 12.49999999999993960, 2.500000000000000000, -4.430127018922202176 ) ) ;
#1009=DIRECTION ( 'NONE',  ( 0.000000000000000000, 0.000000000000000000, -1.000000000000000000 ) ) ;
#1010=VERTEX_POINT ( 'NONE', #35940 ) ;
#1011=CARTESIAN_POINT ( 'NONE',  ( -4.350000000000023626, 2.500000000000000000, -2.511473670974877948 ) ) ;
#1012=EDGE_LOOP ( 'NONE', ( #21519, #20729 ) ) ;
#1013=CONICAL_SURFACE ( 'NONE', #32441, 0.09999999999999982514, 0.003490658503988666988 ) ;
#1014=ORIENTED_EDGE ( 'NONE', *, *, #70820, .T. ) ;
#1015=CARTESIAN_POINT ( 'NONE',  ( -6.650000000000019007, 2.500000000000000000, -5.902370205355750521 ) ) ;
#1016=VECTOR ( 'NONE', #53390, 1000.000000000000000 ) ;
#1017=AXIS2_PLACEMENT_3D ( 'NONE', #89269, #99100, #28425 ) ;
#1018=CARTESIAN_POINT ( 'NONE',  ( -1.650000000000035660, 2.500000000000000000, 7.088010851410848190 ) ) ;
#1019=CARTESIAN_POINT ( 'NONE',  ( -5.850000000000022737, 2.500000000000000000, -6.495190528383302464 ) ) ;
#1020=VERTEX_POINT ( 'NONE', #96143 ) ;
#1021=ORIENTED_EDGE ( 'NONE', *, *, #102730, .F. ) ;
#1022=FACE_OUTER_BOUND ( 'NONE', #57191, .T. ) ;
#1023=CONICAL_SURFACE ( 'NONE', #97171, 0.1000000000000002554, 0.003490658503988666988 ) ;
#1024=EDGE_CURVE ( 'NONE', #126709, #55928, #16911, .T. ) ;
#1025=VECTOR ( 'NONE', #26482, 1000.000000000000000 ) ;
#1026=CARTESIAN_POINT ( 'NONE',  ( 5.399999999999934630, 2.500000000000000000, 0.6928203230275494784 ) ) ;
#1027=DIRECTION ( 'NONE',  ( -4.274815082592931898E-19, -0.9999939076577903929, -0.003490651415223739937 ) ) ;
#1028=DIRECTION ( 'NONE',  ( 0.000000000000000000, 0.000000000000000000, 1.000000000000000000 ) ) ;
#1029=VERTEX_POINT ( 'NONE', #105968 ) ;
#1030=CIRCLE ( 'NONE', #103446, 0.06509327318403745899 ) ;
#1031=DIRECTION ( 'NONE',  ( -0.000000000000000000, 1.000000000000000000, -0.000000000000000000 ) ) ;
#1032=ORIENTED_EDGE ( 'NONE', *, *, #41319, .T. ) ;
#1033=CARTESIAN_POINT ( 'NONE',  ( 12.89999999999989733, 2.500000000000000000, -2.385244779468109755E-15 ) ) ;
#1034=AXIS2_PLACEMENT_3D ( 'NONE', #123543, #109047, #126132 ) ;
#1035=CIRCLE ( 'NONE', #74199, 0.1000000000000000472 ) ;
#1036=EDGE_LOOP ( 'NONE', ( #81475, #129207 ) ) ;
#1037=CARTESIAN_POINT ( 'NONE',  ( 17.50000000000000000, 2.500000000000000000, 3.666666666666666963 ) ) ;
#1038=CARTESIAN_POINT ( 'NONE',  ( 9.149999999999918643, 2.500000000000000000, 2.165063509461097713 ) ) ;
#1039=DIRECTION ( 'NONE',  ( 0.000000000000000000, -0.000000000000000000, 1.000000000000000000 ) ) ;
#1040=CIRCLE ( 'NONE', #78431, 0.1000000000000002554 ) ;
#1041=FACE_OUTER_BOUND ( 'NONE', #46553, .T. ) ;
#1042=EDGE_LOOP ( 'NONE', ( #1365, #8512, #87614, #90230 ) ) ;
#1043=CARTESIAN_POINT ( 'NONE',  ( -13.74999999999995381, 2.500000000000000000, 2.165063509461101265 ) ) ;
#1044=CARTESIAN_POINT ( 'NONE',  ( 8.549999999999924327, 2.500000000000000000, -6.841600689897077814 ) ) ;
#1045=ORIENTED_EDGE ( 'NONE', *, *, #38814, .T. ) ;
#1046=VERTEX_POINT ( 'NONE', #51574 ) ;
#1047=ORIENTED_EDGE ( 'NONE', *, *, #124636, .T. ) ;
#1048=CARTESIAN_POINT ( 'NONE',  ( 2.500000000000002220, -0.9166666666666694052, 10.00000000000000178 ) ) ;
#1049=DIRECTION ( 'NONE',  ( 0.000000000000000000, 0.000000000000000000, 1.000000000000000000 ) ) ;
#1050=CARTESIAN_POINT ( 'NONE',  ( -9.600000000000006750, 12.50000000000000000, 3.637306695894644726 ) ) ;
#1051=CARTESIAN_POINT ( 'NONE',  ( 4.399999999999937295, 2.500000000000000000, 4.083716857408421497 ) ) ;
#1052=AXIS2_PLACEMENT_3D ( 'NONE', #24332, #114006, #43982 ) ;
#1053=CARTESIAN_POINT ( 'NONE',  ( -3.350000000000029399, 2.500000000000000000, 6.495190528383297135 ) ) ;
#1054=FACE_OUTER_BOUND ( 'NONE', #2883, .T. ) ;
#1055=DIRECTION ( 'NONE',  ( 0.000000000000000000, 0.000000000000000000, 1.000000000000000000 ) ) ;
#1056=CARTESIAN_POINT ( 'NONE',  ( -10.00000000000000533, 2.500000000000000000, 5.022947341949748790 ) ) ;
#1057=DIRECTION ( 'NONE',  ( 0.000000000000000000, -0.9999939076577903929, 0.003490651415223739937 ) ) ;
#1058=CONICAL_SURFACE ( 'NONE', #15714, 0.1000000000000002554, 0.003490658503988666988 ) ;
#1059=CIRCLE ( 'NONE', #74226, 0.1000000000000002554 ) ;
#1060=EDGE_CURVE ( 'NONE', #35393, #66105, #46193, .T. ) ;
#1061=VERTEX_POINT ( 'NONE', #71193 ) ;
#1063=ADVANCED_FACE ( 'NONE', ( #50928 ), #6447, .T. ) ;
#1064=DIRECTION ( 'NONE',  ( 0.000000000000000000, 1.000000000000000000, 0.000000000000000000 ) ) ;
#1065=CARTESIAN_POINT ( 'NONE',  ( 1.249999999999954259, 2.500000000000000000, -7.288010851410854585 ) ) ;
#1066=DIRECTION ( 'NONE',  ( -0.000000000000000000, -1.000000000000000000, -0.000000000000000000 ) ) ;
#1067=ADVANCED_FACE ( 'NONE', ( #50277 ), #60866, .T. ) ;
#1068=EDGE_LOOP ( 'NONE', ( #104380, #90932, #57767, #56448 ) ) ;
#1069=DIRECTION ( 'NONE',  ( -0.000000000000000000, 1.000000000000000000, -0.000000000000000000 ) ) ;
#1070=AXIS2_PLACEMENT_3D ( 'NONE', #62806, #33363, #52331 ) ;
#1071=CARTESIAN_POINT ( 'NONE',  ( 0.3999999999999555023, 12.50000000000000000, 4.330127018922196314 ) ) ;
#1072=LINE ( 'NONE', #3653, #31661 ) ;
#1073=ORIENTED_EDGE ( 'NONE', *, *, #100282, .F. ) ;
#1074=EDGE_CURVE ( 'NONE', #58319, #8778, #109867, .T. ) ;
#1075=EDGE_CURVE ( 'NONE', #24109, #85332, #128671, .T. ) ;
#1076=ADVANCED_FACE ( 'NONE', ( #110478 ), #13694, .T. ) ;
#1077=ADVANCED_FACE ( 'NONE', ( #100643 ), #63884, .T. ) ;
#1078=EDGE_CURVE ( 'NONE', #3798, #21836, #99406, .T. ) ;
#1079=EDGE_LOOP ( 'NONE', ( #32587, #83909 ) ) ;
#1080=CARTESIAN_POINT ( 'NONE',  ( 2.499999999999947153, 2.500000000000000000, 0.6928203230275494784 ) ) ;
#1081=AXIS2_PLACEMENT_3D ( 'NONE', #63126, #90652, #80846 ) ;
#1083=EDGE_LOOP ( 'NONE', ( #127551, #120321, #103737, #57132 ) ) ;
#1084=FACE_OUTER_BOUND ( 'NONE', #30197, .T. ) ;
#1085=EDGE_CURVE ( 'NONE', #94776, #42733, #101315, .T. ) ;
#1086=CARTESIAN_POINT ( 'NONE',  ( 21.24754738303297330, 0.7337760880902505223, -4.182111650399365388 ) ) ;
#1087=CARTESIAN_POINT ( 'NONE',  ( 11.04999999999991012, 2.500000000000000000, 6.841600689897072485 ) ) ;
#1088=DIRECTION ( 'NONE',  ( 0.000000000000000000, 0.000000000000000000, 1.000000000000000000 ) ) ;
#1089=EDGE_CURVE ( 'NONE', #123569, #92739, #5286, .T. ) ;
#1090=ORIENTED_EDGE ( 'NONE', *, *, #103759, .F. ) ;
#1091=FACE_OUTER_BOUND ( 'NONE', #74753, .T. ) ;
#1092=ORIENTED_EDGE ( 'NONE', *, *, #21775, .T. ) ;
#1093=CARTESIAN_POINT ( 'NONE',  ( -5.400000000000019895, 2.500000000000000000, -0.7928203230275542301 ) ) ;
#1094=SHAPE_REPRESENTATION ( 'Brush Head Assembly', ( #108296 ), #79070 ) ;
#1095=DIRECTION ( 'NONE',  ( 0.000000000000000000, 1.000000000000000000, 0.000000000000000000 ) ) ;
#1096=VECTOR ( 'NONE', #95538, 1000.000000000000000 ) ;
#1097=ORIENTED_EDGE ( 'NONE', *, *, #54469, .T. ) ;
#1099=CIRCLE ( 'NONE', #95207, 0.09999999999999982514 ) ;
#1100=ORIENTED_EDGE ( 'NONE', *, *, #118125, .F. ) ;
#1101=ORIENTED_EDGE ( 'NONE', *, *, #20054, .T. ) ;
#1102=FACE_OUTER_BOUND ( 'NONE', #310, .T. ) ;
#1103=CARTESIAN_POINT ( 'NONE',  ( 10.30524027341048843, 2.500000000000255795, 9.130939513283916398 ) ) ;
#1104=AXIS2_PLACEMENT_3D ( 'NONE', #80551, #17737, #87765 ) ;
#1105=PLANE ( 'NONE',  #100600 ) ;
#1106=FACE_BOUND ( 'NONE', #107447, .T. ) ;
#1107=DIRECTION ( 'NONE',  ( 0.000000000000000000, 0.000000000000000000, -1.000000000000000000 ) ) ;
#1109=DIRECTION ( 'NONE',  ( 0.000000000000000000, 0.000000000000000000, 1.000000000000000000 ) ) ;
#1110=DIRECTION ( 'NONE',  ( 0.000000000000000000, 0.000000000000000000, -1.000000000000000000 ) ) ;
#1112=AXIS2_PLACEMENT_3D ( 'NONE', #31334, #127742, #46602 ) ;
#1113=FACE_OUTER_BOUND ( 'NONE', #44992, .T. ) ;
#1114=AXIS2_PLACEMENT_3D ( 'NONE', #95902, #65786, #78208 ) ;
#1115=LINE ( 'NONE', #3693, #7032 ) ;
#1116=ADVANCED_FACE ( 'NONE', ( #41119 ), #32516, .T. ) ;
#1118=EDGE_CURVE ( 'NONE', #65792, #60753, #101952, .T. ) ;
#1119=AXIS2_PLACEMENT_3D ( 'NONE', #101193, #111660, #90723 ) ;
#1120=CONICAL_SURFACE ( 'NONE', #78516, 0.1000000000000002554, 0.003490658503988666988 ) ;
#1121=DIRECTION ( 'NONE',  ( 0.000000000000000000, 0.000000000000000000, 1.000000000000000000 ) ) ;
#1122=EDGE_CURVE ( 'NONE', #21908, #57789, #128863, .T. ) ;
#1123=ORIENTED_EDGE ( 'NONE', *, *, #105248, .F. ) ;
#1124=VERTEX_POINT ( 'NONE', #39191 ) ;
#1125=VERTEX_POINT ( 'NONE', #1800 ) ;
#1126=EDGE_LOOP ( 'NONE', ( #75811, #97863 ) ) ;
#1127=AXIS2_PLACEMENT_3D ( 'NONE', #59022, #38766, #108112 ) ;
#1128=ORIENTED_EDGE ( 'NONE', *, *, #63191, .F. ) ;
#1129=DIRECTION ( 'NONE',  ( 0.000000000000000000, 1.000000000000000000, 0.000000000000000000 ) ) ;
#1130=DIRECTION ( 'NONE',  ( -0.000000000000000000, -1.000000000000000000, -0.000000000000000000 ) ) ;
#1132=EDGE_CURVE ( 'NONE', #88013, #108519, #103610, .T. ) ;
#1133=FACE_BOUND ( 'NONE', #57001, .T. ) ;
#1134=DIRECTION ( 'NONE',  ( 0.000000000000000000, 0.000000000000000000, 1.000000000000000000 ) ) ;
#1135=ADVANCED_FACE ( 'NONE', ( #121576 ), #88934, .T. ) ;
#1137=ORIENTED_EDGE ( 'NONE', *, *, #42942, .T. ) ;
#1138=DIRECTION ( 'NONE',  ( -0.000000000000000000, -1.000000000000000000, -0.000000000000000000 ) ) ;
#1140=CARTESIAN_POINT ( 'NONE',  ( 8.749999999999953815, 2.500000000000000000, 6.595190528383296780 ) ) ;
#1141=CARTESIAN_POINT ( 'NONE',  ( -8.950000000000006395, 12.50000000000000000, 6.841600689897072485 ) ) ;
#1142=AXIS2_PLACEMENT_3D ( 'NONE', #35448, #115249, #27529 ) ;
#1143=ORIENTED_EDGE ( 'NONE', *, *, #102989, .F. ) ;
#1144=DIRECTION ( 'NONE',  ( 0.000000000000000000, 1.000000000000000000, 0.000000000000000000 ) ) ;
#1145=ADVANCED_FACE ( 'NONE', ( #59478 ), #36711, .T. ) ;
#1146=EDGE_LOOP ( 'NONE', ( #88682, #16117 ) ) ;
#1147=ORIENTED_EDGE ( 'NONE', *, *, #35573, .F. ) ;
#1148=CARTESIAN_POINT ( 'NONE',  ( -5.600000000000020073, 12.50000000000000000, 4.676537180435972552 ) ) ;
#1149=CARTESIAN_POINT ( 'NONE',  ( -1.250000000000036193, 2.500000000000000000, 5.802370205355744659 ) ) ;
#1150=AXIS2_PLACEMENT_3D ( 'NONE', #42717, #70863, #110771 ) ;
#1151=ORIENTED_EDGE ( 'NONE', *, *, #63327, .F. ) ;
#1152=DIRECTION ( 'NONE',  ( 0.000000000000000000, 0.000000000000000000, 1.000000000000000000 ) ) ;
#1153=AXIS2_PLACEMENT_3D ( 'NONE', #77461, #118027, #89218 ) ;
#1154=AXIS2_PLACEMENT_3D ( 'NONE', #37682, #78907, #89983 ) ;
#1155=FACE_OUTER_BOUND ( 'NONE', #34928, .T. ) ;
#1156=DIRECTION ( 'NONE',  ( 0.000000000000000000, 0.000000000000000000, 1.000000000000000000 ) ) ;
#1157=CARTESIAN_POINT ( 'NONE',  ( -6.650000000000018119, 12.50000000000000000, -2.857883832488653741 ) ) ;
#1158=EDGE_LOOP ( 'NONE', ( #77071, #69585 ) ) ;
#1159=FACE_OUTER_BOUND ( 'NONE', #85226, .T. ) ;
#1160=EDGE_CURVE ( 'NONE', #14447, #93919, #13555, .T. ) ;
#1161=ORIENTED_EDGE ( 'NONE', *, *, #44076, .T. ) ;
#1162=DIRECTION ( 'NONE',  ( 1.000000000000000000, 0.000000000000000000, 0.000000000000000000 ) ) ;
#1163=CIRCLE ( 'NONE', #26314, 0.06509327318403745899 ) ;
#1164=ORIENTED_EDGE ( 'NONE', *, *, #15453, .F. ) ;
#1165=AXIS2_PLACEMENT_3D ( 'NONE', #71829, #42368, #100001 ) ;
#1166=FACE_OUTER_BOUND ( 'NONE', #110008, .T. ) ;
#1167=ORIENTED_EDGE ( 'NONE', *, *, #16843, .F. ) ;
#1168=CARTESIAN_POINT ( 'NONE',  ( -6.650000000000018119, 2.500000000000000000, -7.188010851410854052 ) ) ;
#1169=DIRECTION ( 'NONE',  ( 0.000000000000000000, 0.000000000000000000, -1.000000000000000000 ) ) ;
#1170=DIRECTION ( 'NONE',  ( 0.000000000000000000, -0.000000000000000000, 1.000000000000000000 ) ) ;
#1171=DIRECTION ( 'NONE',  ( 0.000000000000000000, 0.000000000000000000, 1.000000000000000000 ) ) ;
#1172=LINE ( 'NONE', #41123, #72590 ) ;
#1173=ORIENTED_EDGE ( 'NONE', *, *, #88308, .T. ) ;
#1174=ORIENTED_EDGE ( 'NONE', *, *, #19, .F. ) ;
#1175=ORIENTED_EDGE ( 'NONE', *, *, #113846, .T. ) ;
#1176=CARTESIAN_POINT ( 'NONE',  ( -2.900000000000029665, 2.500000000000000000, 4.330127018922196314 ) ) ;
#1177=AXIS2_PLACEMENT_3D ( 'NONE', #78084, #89190, #49287 ) ;
#1178=CIRCLE ( 'NONE', #17897, 0.1000000000000002554 ) ;
#1179=EDGE_CURVE ( 'NONE', #106389, #62016, #63962, .T. ) ;
#1180=CARTESIAN_POINT ( 'NONE',  ( 9.149999999999920419, 2.500000000000000000, -7.188010851410854052 ) ) ;
#1181=CARTESIAN_POINT ( 'NONE',  ( -4.076600168545496672E-14, 2.500000000000000000, -5.022947341949754119 ) ) ;
#1182=ORIENTED_EDGE ( 'NONE', *, *, #89891, .T. ) ;
#1183=VERTEX_POINT ( 'NONE', #84228 ) ;
#1184=VERTEX_POINT ( 'NONE', #73137 ) ;
#1185=DIRECTION ( 'NONE',  ( -0.000000000000000000, -1.000000000000000000, -0.000000000000000000 ) ) ;
#1186=EDGE_LOOP ( 'NONE', ( #60111, #65298, #25080, #7290 ) ) ;
#1187=FACE_OUTER_BOUND ( 'NONE', #64228, .T. ) ;
#1188=DIRECTION ( 'NONE',  ( 0.000000000000000000, 0.000000000000000000, 1.000000000000000000 ) ) ;
#1189=LINE ( 'NONE', #41141, #11390 ) ;
#1190=FACE_OUTER_BOUND ( 'NONE', #75353, .T. ) ;
#1191=CARTESIAN_POINT ( 'NONE',  ( -3.100000000000028955, 2.500000000000000000, 3.983716857408420964 ) ) ;
#1192=DIRECTION ( 'NONE',  ( -0.000000000000000000, 1.000000000000000000, -0.000000000000000000 ) ) ;
#1193=DIRECTION ( 'NONE',  ( 0.000000000000000000, 0.000000000000000000, 1.000000000000000000 ) ) ;
#1194=ADVANCED_FACE ( 'NONE', ( #12897 ), #72503, .T. ) ;
#1195=AXIS2_PLACEMENT_3D ( 'NONE', #81684, #121600, #69941 ) ;
#1196=CARTESIAN_POINT ( 'NONE',  ( 8.149999999999923972, 12.50000000000000000, -6.083687093685488989 ) ) ;
#1197=VERTEX_POINT ( 'NONE', #32595 ) ;
#1198=CARTESIAN_POINT ( 'NONE',  ( -10.40000000000000213, 2.500000000000000000, -0.6928203230275541413 ) ) ;
#1199=AXIS2_PLACEMENT_3D ( 'NONE', #76823, #58489, #116728 ) ;
#1200=CIRCLE ( 'NONE', #17920, 0.06509327318403745899 ) ;
#1201=FACE_OUTER_BOUND ( 'NONE', #56405, .T. ) ;
#1202=ORIENTED_EDGE ( 'NONE', *, *, #126692, .T. ) ;
#1203=ORIENTED_EDGE ( 'NONE', *, *, #12560, .T. ) ;
#1205=DIRECTION ( 'NONE',  ( 0.000000000000000000, 0.000000000000000000, -1.000000000000000000 ) ) ;
#1206=DIRECTION ( 'NONE',  ( 0.000000000000000000, 0.000000000000000000, 1.000000000000000000 ) ) ;
#1208=AXIS2_PLACEMENT_3D ( 'NONE', #111977, #40014, #51132 ) ;
#1209=FACE_OUTER_BOUND ( 'NONE', #113304, .T. ) ;
#1210=CARTESIAN_POINT ( 'NONE',  ( -4.800000000000022915, 2.500000000000000000, -0.3464101615137783474 ) ) ;
#1211=CARTESIAN_POINT ( 'NONE',  ( 5.849999999999935696, 2.500000000000000000, -7.088010851410853519 ) ) ;
#1212=CARTESIAN_POINT ( 'NONE',  ( 4.399999999999939071, 2.500000000000000000, -0.4464101615137782142 ) ) ;
#1213=CIRCLE ( 'NONE', #68098, 0.06509327318403745899 ) ;
#1214=CARTESIAN_POINT ( 'NONE',  ( -1.250000000000036193, 2.500000000000000000, 1.472243186433545459 ) ) ;
#1215=VECTOR ( 'NONE', #47434, 1000.000000000000000 ) ;
#1216=CONICAL_SURFACE ( 'NONE', #40959, 0.09999999999999982514, 0.003490658503988666988 ) ;
#1217=ORIENTED_EDGE ( 'NONE', *, *, #56795, .F. ) ;
#1218=ORIENTED_EDGE ( 'NONE', *, *, #101381, .T. ) ;
#1219=VECTOR ( 'NONE', #63000, 1000.000000000000000 ) ;
#1220=ADVANCED_FACE ( 'NONE', ( #43062 ), #45026, .T. ) ;
#1221=ORIENTED_EDGE ( 'NONE', *, *, #45182, .T. ) ;
#1222=ORIENTED_EDGE ( 'NONE', *, *, #15384, .T. ) ;
#1223=ORIENTED_EDGE ( 'NONE', *, *, #53101, .F. ) ;
#1224=PLANE ( 'NONE',  #42103 ) ;
#1225=FACE_OUTER_BOUND ( 'NONE', #37159, .T. ) ;
#1227=ORIENTED_EDGE ( 'NONE', *, *, #26923, .T. ) ;
#1228=DIRECTION ( 'NONE',  ( 0.000000000000000000, 1.000000000000000000, 0.000000000000000000 ) ) ;
#1229=DIRECTION ( 'NONE',  ( 0.000000000000000000, 1.000000000000000000, 0.000000000000000000 ) ) ;
#1230=CARTESIAN_POINT ( 'NONE',  ( 10.84999999999991260, 2.500000000000000000, 5.802370205355744659 ) ) ;
#1231=DIRECTION ( 'NONE',  ( 0.000000000000000000, 0.000000000000000000, 1.000000000000000000 ) ) ;
#1232=EDGE_LOOP ( 'NONE', ( #95732, #16124 ) ) ;
#1233=EDGE_CURVE ( 'NONE', #62826, #110935, #84883, .T. ) ;
#1234=ADVANCED_FACE ( 'NONE', ( #52209 ), #65230, .T. ) ;
#1235=EDGE_CURVE ( 'NONE', #53159, #69354, #47167, .T. ) ;
#1236=CARTESIAN_POINT ( 'NONE',  ( 8.099999999999923261, 2.500000000000000000, -4.776537180435978414 ) ) ;
#1237=EDGE_CURVE ( 'NONE', #120782, #8397, #7439, .T. ) ;
#1238=CIRCLE ( 'NONE', #126639, 0.06509327318403745899 ) ;
#1239=FACE_OUTER_BOUND ( 'NONE', #8734, .T. ) ;
#1240=ORIENTED_EDGE ( 'NONE', *, *, #56224, .T. ) ;
#1241=ADVANCED_FACE ( 'NONE', ( #35162 ), #95192, .T. ) ;
#1242=ORIENTED_EDGE ( 'NONE', *, *, #51274, .F. ) ;
#1243=EDGE_LOOP ( 'NONE', ( #124951, #37318 ) ) ;
#1244=ORIENTED_EDGE ( 'NONE', *, *, #100146, .F. ) ;
#1245=DIRECTION ( 'NONE',  ( 0.000000000000000000, 0.000000000000000000, 1.000000000000000000 ) ) ;
#1246=EDGE_CURVE ( 'NONE', #105517, #83506, #22043, .T. ) ;
#1247=VECTOR ( 'NONE', #117999, 1000.000000000000000 ) ;
#1248=CARTESIAN_POINT ( 'NONE',  ( 4.799999999999935874, 2.500000000000000000, 0.3464101615137735735 ) ) ;
#1249=CARTESIAN_POINT ( 'NONE',  ( 2.500000000000002220, -2.500000000000000000, -9.261799387799147354 ) ) ;
#1250=AXIS2_PLACEMENT_3D ( 'NONE', #108337, #88029, #118162 ) ;
#1251=EDGE_CURVE ( 'NONE', #4623, #7925, #55483, .T. ) ;
#1252=ADVANCED_FACE ( 'NONE', ( #44974 ), #23568, .T. ) ;
#1253=CIRCLE ( 'NONE', #74415, 0.06509327318403745899 ) ;
#1255=VERTEX_POINT ( 'NONE', #54770 ) ;
#1256=CARTESIAN_POINT ( 'NONE',  ( 13.74999999999989875, 12.50000000000000000, 1.472243186433545459 ) ) ;
#1257=LINE ( 'NONE', #41204, #120746 ) ;
#1258=CARTESIAN_POINT ( 'NONE',  ( -7.700000000000010836, 12.50000000000000000, 3.983716857408420964 ) ) ;
#1259=CARTESIAN_POINT ( 'NONE',  ( 9.199999999999915801, 2.500000000000000000, -4.330127018922201643 ) ) ;
#1260=EDGE_CURVE ( 'NONE', #129522, #47326, #73726, .T. ) ;
#1261=CIRCLE ( 'NONE', #68150, 0.06509327318403745899 ) ;
#1262=VERTEX_POINT ( 'NONE', #122886 ) ;
#1263=VECTOR ( 'NONE', #94221, 1000.000000000000000 ) ;
#1264=ORIENTED_EDGE ( 'NONE', *, *, #70825, .F. ) ;
#1265=VERTEX_POINT ( 'NONE', #25298 ) ;
#1266=DIRECTION ( 'NONE',  ( 0.000000000000000000, -0.000000000000000000, 1.000000000000000000 ) ) ;
#1267=LINE ( 'NONE', #3840, #114989 ) ;
#1268=FACE_BOUND ( 'NONE', #43258, .T. ) ;
#1269=DIRECTION ( 'NONE',  ( -0.000000000000000000, 1.000000000000000000, -0.000000000000000000 ) ) ;
#1270=CARTESIAN_POINT ( 'NONE',  ( -7.050000000000016698, 2.500000000000000000, -2.165063509461101710 ) ) ;
#1271=FACE_OUTER_BOUND ( 'NONE', #75762, .T. ) ;
#1272=AXIS2_PLACEMENT_3D ( 'NONE', #26918, #47859, #17054 ) ;
#1273=DIRECTION ( 'NONE',  ( 0.000000000000000000, 1.000000000000000000, 0.000000000000000000 ) ) ;
#1274=CARTESIAN_POINT ( 'NONE',  ( -12.69999999999999218, 12.50000000000000000, 4.676537180435972552 ) ) ;
#1275=FACE_OUTER_BOUND ( 'NONE', #100380, .T. ) ;
#1276=ORIENTED_EDGE ( 'NONE', *, *, #2567, .T. ) ;
#1277=FACE_OUTER_BOUND ( 'NONE', #39005, .T. ) ;
#1278=CARTESIAN_POINT ( 'NONE',  ( 6.849999999999930367, 12.50000000000000000, -6.776507416713040577 ) ) ;
#1279=ORIENTED_EDGE ( 'NONE', *, *, #7307, .T. ) ;
#1280=EDGE_LOOP ( 'NONE', ( #1759, #3092, #98830, #88037 ) ) ;
#1281=DIRECTION ( 'NONE',  ( 0.000000000000000000, 0.000000000000000000, 1.000000000000000000 ) ) ;
#1282=CARTESIAN_POINT ( 'NONE',  ( 10.84999999999990905, 2.500000000000000000, -7.288010851410854585 ) ) ;
#1283=FACE_BOUND ( 'NONE', #29371, .T. ) ;
#1284=DIRECTION ( 'NONE',  ( -0.000000000000000000, 1.000000000000000000, -0.000000000000000000 ) ) ;
#1285=EDGE_CURVE ( 'NONE', #65003, #93435, #96710, .T. ) ;
#1286=CONICAL_SURFACE ( 'NONE', #7534, 0.09999999999999982514, 0.003490658503988666988 ) ;
#1287=LINE ( 'NONE', #60239, #54902 ) ;
#1288=EDGE_CURVE ( 'NONE', #110742, #77067, #67759, .T. ) ;
#1289=ORIENTED_EDGE ( 'NONE', *, *, #26689, .F. ) ;
#1290=LINE ( 'NONE', #22241, #2696 ) ;
#1291=CARTESIAN_POINT ( 'NONE',  ( 1.249999999999988454, 12.50000000000000000, 2.165063509461097713 ) ) ;
#1292=VERTEX_POINT ( 'NONE', #3113 ) ;
#1293=DIRECTION ( 'NONE',  ( -0.000000000000000000, -1.000000000000000000, -0.000000000000000000 ) ) ;
#1294=FACE_OUTER_BOUND ( 'NONE', #121910, .T. ) ;
#1295=EDGE_CURVE ( 'NONE', #118275, #98777, #128552, .T. ) ;
#1296=CIRCLE ( 'NONE', #43377, 0.09999999999999982514 ) ;
#1297=VECTOR ( 'NONE', #4974, 1000.000000000000000 ) ;
#1298=DIRECTION ( 'NONE',  ( 0.000000000000000000, 0.000000000000000000, 1.000000000000000000 ) ) ;
#1299=PLANE ( 'NONE',  #126302 ) ;
#1300=CIRCLE ( 'NONE', #97452, 0.06509327318403745899 ) ;
#1301=CIRCLE ( 'NONE', #116310, 0.06509327318403745899 ) ;
#1302=ORIENTED_EDGE ( 'NONE', *, *, #63770, .T. ) ;
#1303=AXIS2_PLACEMENT_3D ( 'NONE', #65571, #46568, #38054 ) ;
#1304=DIRECTION ( 'NONE',  ( 0.000000000000000000, 0.000000000000000000, -1.000000000000000000 ) ) ;
#1305=CARTESIAN_POINT ( 'NONE',  ( -2.900000000000029665, 2.500000000000000000, 3.637306695894644726 ) ) ;
#1306=DIRECTION ( 'NONE',  ( 0.000000000000000000, 0.000000000000000000, -1.000000000000000000 ) ) ;
#1308=ORIENTED_EDGE ( 'NONE', *, *, #106310, .T. ) ;
#1309=FACE_OUTER_BOUND ( 'NONE', #46149, .T. ) ;
#1310=ORIENTED_EDGE ( 'NONE', *, *, #78972, .F. ) ;
#1311=DIRECTION ( 'NONE',  ( 0.000000000000000000, 0.000000000000000000, 1.000000000000000000 ) ) ;
#1312=LINE ( 'NONE', #113194, #30722 ) ;
#1313=CARTESIAN_POINT ( 'NONE',  ( 4.399999999999937295, 2.500000000000000000, 3.983716857408420964 ) ) ;
#1314=VERTEX_POINT ( 'NONE', #49986 ) ;
#1315=DIRECTION ( 'NONE',  ( -0.000000000000000000, 1.000000000000000000, -0.000000000000000000 ) ) ;
#1316=CARTESIAN_POINT ( 'NONE',  ( 2.699999999999946443, 12.50000000000000000, 0.3464101615137735735 ) ) ;
#1317=DIRECTION ( 'NONE',  ( 0.000000000000000000, -0.9999939076577903929, 0.003490651415223739937 ) ) ;
#1318=DIRECTION ( 'NONE',  ( 0.000000000000000000, 0.000000000000000000, -1.000000000000000000 ) ) ;
#1319=DIRECTION ( 'NONE',  ( 0.000000000000000000, 0.000000000000000000, 1.000000000000000000 ) ) ;
#1320=CIRCLE ( 'NONE', #36847, 0.1000000000000000472 ) ;
#1321=DIRECTION ( 'NONE',  ( 0.000000000000000000, 0.000000000000000000, 1.000000000000000000 ) ) ;
#1322=ORIENTED_EDGE ( 'NONE', *, *, #125991, .F. ) ;
#1323=ORIENTED_EDGE ( 'NONE', *, *, #22673, .F. ) ;
#1324=DIRECTION ( 'NONE',  ( 0.000000000000000000, 1.000000000000000000, 0.000000000000000000 ) ) ;
#1325=ORIENTED_EDGE ( 'NONE', *, *, #65628, .T. ) ;
#1326=AXIS2_PLACEMENT_3D ( 'NONE', #104398, #63835, #72374 ) ;
#1328=ORIENTED_EDGE ( 'NONE', *, *, #113030, .F. ) ;
#1329=EDGE_LOOP ( 'NONE', ( #53660, #26725 ) ) ;
#1330=AXIS2_PLACEMENT_3D ( 'NONE', #86304, #57514, #117044 ) ;
#1331=EDGE_LOOP ( 'NONE', ( #72263, #28879, #15786, #82302 ) ) ;
#1332=CARTESIAN_POINT ( 'NONE',  ( 8.349999999999923261, 12.50000000000000000, 2.099970236277060032 ) ) ;
#1333=VECTOR ( 'NONE', #38513, 1000.000000000000000 ) ;
#1334=AXIS2_PLACEMENT_3D ( 'NONE', #20461, #101598, #10607 ) ;
#1335=CARTESIAN_POINT ( 'NONE',  ( -1.450000000000036371, 2.500000000000000000, 6.841600689897072485 ) ) ;
#1336=DIRECTION ( 'NONE',  ( 0.000000000000000000, 1.000000000000000000, 0.000000000000000000 ) ) ;
#1337=CARTESIAN_POINT ( 'NONE',  ( -0.8000000000000315747, 2.500000000000000000, 0.000000000000000000 ) ) ;
#1338=DIRECTION ( 'NONE',  ( 0.000000000000000000, 0.000000000000000000, -1.000000000000000000 ) ) ;
#1339=CARTESIAN_POINT ( 'NONE',  ( 3.549999999999944755, 2.500000000000000000, -6.841600689897077814 ) ) ;
#1340=EDGE_CURVE ( 'NONE', #2601, #71725, #123903, .T. ) ;
#1341=CARTESIAN_POINT ( 'NONE',  ( -3.350000000000028511, 12.50000000000000000, -2.857883832488653741 ) ) ;
#1342=CARTESIAN_POINT ( 'NONE',  ( -1.900000000000034106, 2.500000000000000000, 0.4464101615137735513 ) ) ;
#1343=ADVANCED_FACE ( 'NONE', ( #70250 ), #124200, .T. ) ;
#1344=DIRECTION ( 'NONE',  ( 0.000000000000000000, 1.000000000000000000, 0.000000000000000000 ) ) ;
#1345=CIRCLE ( 'NONE', #59970, 0.06509327318403745899 ) ;
#1346=ORIENTED_EDGE ( 'NONE', *, *, #57071, .F. ) ;
#1348=CIRCLE ( 'NONE', #55730, 0.1000000000000002554 ) ;
#1349=DIRECTION ( 'NONE',  ( -0.000000000000000000, -1.000000000000000000, -0.000000000000000000 ) ) ;
#1350=VERTEX_POINT ( 'NONE', #108865 ) ;
#1351=EDGE_CURVE ( 'NONE', #25898, #31429, #87294, .T. ) ;
#1352=ORIENTED_EDGE ( 'NONE', *, *, #91149, .T. ) ;
#1354=CARTESIAN_POINT ( 'NONE',  ( 10.84999999999991260, 12.50000000000000000, 6.495190528383297135 ) ) ;
#1355=FACE_OUTER_BOUND ( 'NONE', #119817, .T. ) ;
#1356=CARTESIAN_POINT ( 'NONE',  ( -2.900000000000029221, 12.50000000000000000, -0.6928203230275541413 ) ) ;
#1357=CARTESIAN_POINT ( 'NONE',  ( -9.800000000000006040, 2.500000000000000000, -4.676537180435974328 ) ) ;
#1358=FACE_OUTER_BOUND ( 'NONE', #50552, .T. ) ;
#1359=ORIENTED_EDGE ( 'NONE', *, *, #63750, .T. ) ;
#1360=EDGE_LOOP ( 'NONE', ( #49377, #81992, #122314 ) ) ;
#1361=VERTEX_POINT ( 'NONE', #127245 ) ;
#1362=FACE_OUTER_BOUND ( 'NONE', #11330, .T. ) ;
#1363=ADVANCED_FACE ( 'NONE', ( #59151 ), #119338, .T. ) ;
#1364=ORIENTED_EDGE ( 'NONE', *, *, #72648, .F. ) ;
#1365=ORIENTED_EDGE ( 'NONE', *, *, #24267, .F. ) ;
#1366=DIRECTION ( 'NONE',  ( -0.000000000000000000, -1.000000000000000000, -0.000000000000000000 ) ) ;
#1367=DIRECTION ( 'NONE',  ( 0.000000000000000000, 0.000000000000000000, 1.000000000000000000 ) ) ;
#1368=EDGE_CURVE ( 'NONE', #120113, #49114, #80068, .T. ) ;
#1369=AXIS2_PLACEMENT_3D ( 'NONE', #11132, #61553, #12426 ) ;
#1370=DIRECTION ( 'NONE',  ( -0.000000000000000000, 1.000000000000000000, -0.000000000000000000 ) ) ;
#1371=CIRCLE ( 'NONE', #74543, 0.09999999999999982514 ) ;
#1372=CARTESIAN_POINT ( 'NONE',  ( -12.49999999999995737, 2.500000000000000000, 4.330127018922196314 ) ) ;
#1373=CARTESIAN_POINT ( 'NONE',  ( 17.50000000000000000, -1.666666666666667851, 4.000000000000001776 ) ) ;
#1374=VERTEX_POINT ( 'NONE', #30344 ) ;
#1375=CARTESIAN_POINT ( 'NONE',  ( 4.349999999999941025, 2.500000000000000000, -6.048780366869526581 ) ) ;
#1376=CARTESIAN_POINT ( 'NONE',  ( -12.04999999999999538, 2.500000000000000000, 2.065063509461097624 ) ) ;
#1378=EDGE_CURVE ( 'NONE', #32526, #19824, #107178, .T. ) ;
#1379=CARTESIAN_POINT ( 'NONE',  ( 10.84999999999990905, 2.500000000000000000, -7.188010851410854052 ) ) ;
#1380=EDGE_CURVE ( 'NONE', #50137, #26812, #566, .T. ) ;
#1381=CARTESIAN_POINT ( 'NONE',  ( 10.84999999999991260, 2.500000000000000000, -2.957883832488653830 ) ) ;
#1382=EDGE_CURVE ( 'NONE', #66554, #27692, #120003, .T. ) ;
#1383=AXIS2_PLACEMENT_3D ( 'NONE', #122480, #63559, #123118 ) ;
#1384=CONICAL_SURFACE ( 'NONE', #30660, 0.1000000000000002554, 0.003490658503988666988 ) ;
#1385=DIRECTION ( 'NONE',  ( 0.000000000000000000, 0.000000000000000000, 1.000000000000000000 ) ) ;
#1387=EDGE_LOOP ( 'NONE', ( #28668, #87934 ) ) ;
#1388=ADVANCED_FACE ( 'NONE', ( #5661 ), #113747, .T. ) ;
#1389=EDGE_LOOP ( 'NONE', ( #22240, #45904, #119155, #304 ) ) ;
#1390=DIRECTION ( 'NONE',  ( 0.000000000000000000, 0.000000000000000000, 1.000000000000000000 ) ) ;
#1391=ADVANCED_FACE ( 'NONE', ( #58515 ), #117623, .T. ) ;
#1393=AXIS2_PLACEMENT_3D ( 'NONE', #74636, #111998, #3959 ) ;
#1394=FACE_OUTER_BOUND ( 'NONE', #6170, .T. ) ;
#1395=DIRECTION ( 'NONE',  ( 0.000000000000000000, 0.000000000000000000, -1.000000000000000000 ) ) ;
#1396=EDGE_CURVE ( 'NONE', #59296, #94218, #34037, .T. ) ;
#1397=ADVANCED_FACE ( 'NONE', ( #107594 ), #84193, .T. ) ;
#1398=EDGE_LOOP ( 'NONE', ( #37016, #92349 ) ) ;
#1399=FACE_OUTER_BOUND ( 'NONE', #32904, .T. ) ;
#1400=DIRECTION ( 'NONE',  ( 0.000000000000000000, 1.000000000000000000, 0.000000000000000000 ) ) ;
#1401=EDGE_CURVE ( 'NONE', #83172, #54921, #74024, .T. ) ;
#1402=CARTESIAN_POINT ( 'NONE',  ( -12.94999999999999218, 2.500000000000000000, -2.165063509461099489 ) ) ;
#1403=CARTESIAN_POINT ( 'NONE',  ( 14.34999999999989662, 2.500000000000000000, 2.411473670974873862 ) ) ;
#1404=ADVANCED_FACE ( 'NONE', ( #99070 ), #28396, .T. ) ;
#1405=DIRECTION ( 'NONE',  ( 0.000000000000000000, 1.000000000000000000, 0.000000000000000000 ) ) ;
#1406=VERTEX_POINT ( 'NONE', #48679 ) ;
#1407=ORIENTED_EDGE ( 'NONE', *, *, #69792, .F. ) ;
#1408=LINE ( 'NONE', #59721, #100806 ) ;
#1409=CIRCLE ( 'NONE', #128988, 0.06509327318403745899 ) ;
#1411=AXIS2_PLACEMENT_3D ( 'NONE', #95661, #26921, #115942 ) ;
#1412=CARTESIAN_POINT ( 'NONE',  ( -9.600000000000008527, 12.50000000000000000, -4.330127018922197202 ) ) ;
#1413=DIRECTION ( 'NONE',  ( -0.000000000000000000, 1.000000000000000000, -0.000000000000000000 ) ) ;
#1414=ORIENTED_EDGE ( 'NONE', *, *, #64492, .T. ) ;
#1415=AXIS2_PLACEMENT_3D ( 'NONE', #22542, #51359, #62463 ) ;
#1416=ORIENTED_EDGE ( 'NONE', *, *, #126850, .F. ) ;
#1417=LINE ( 'NONE', #79984, #45970 ) ;
#1418=DIRECTION ( 'NONE',  ( 0.000000000000000000, 1.000000000000000000, 0.000000000000000000 ) ) ;
#1419=AXIS2_PLACEMENT_3D ( 'NONE', #65191, #103861, #123481 ) ;
#1420=CARTESIAN_POINT ( 'NONE',  ( 8.349999999999919709, 2.500000000000000000, -1.572243186433550211 ) ) ;
#1421=CIRCLE ( 'NONE', #53663, 0.06509327318403745899 ) ;
#1423=DIRECTION ( 'NONE',  ( -0.000000000000000000, 1.000000000000000000, -0.000000000000000000 ) ) ;
#1424=VECTOR ( 'NONE', #85113, 1000.000000000000000 ) ;
#1425=DIRECTION ( 'NONE',  ( 0.000000000000000000, 1.000000000000000000, 0.000000000000000000 ) ) ;
#1426=ORIENTED_EDGE ( 'NONE', *, *, #123113, .T. ) ;
#1427=CARTESIAN_POINT ( 'NONE',  ( -2.700000000000029932, 2.500000000000000000, -4.676537180435977881 ) ) ;
#1428=EDGE_LOOP ( 'NONE', ( #20451, #119614 ) ) ;
#1429=CIRCLE ( 'NONE', #51631, 0.06509327318403745899 ) ;
#1431=ORIENTED_EDGE ( 'NONE', *, *, #49770, .T. ) ;
#1432=ADVANCED_FACE ( 'NONE', ( #79438 ), #869, .T. ) ;
#1433=VECTOR ( 'NONE', #68469, 1000.000000000000000 ) ;
#1434=CIRCLE ( 'NONE', #59973, 0.06509327318403745899 ) ;
#1435=VERTEX_POINT ( 'NONE', #1495 ) ;
#1436=CARTESIAN_POINT ( 'NONE',  ( -8.150000000000012790, 12.50000000000000000, -2.511473670974877948 ) ) ;
#1437=CARTESIAN_POINT ( 'NONE',  ( 3.299999999999944755, 2.500000000000000000, -4.330127018922201643 ) ) ;
#1438=ADVANCED_FACE ( 'NONE', ( #51907 ), #34338, .T. ) ;
#1439=ORIENTED_EDGE ( 'NONE', *, *, #63482, .T. ) ;
#1440=EDGE_LOOP ( 'NONE', ( #100464, #41406 ) ) ;
#1441=CARTESIAN_POINT ( 'NONE',  ( 4.149999999999941735, 2.500000000000000000, -1.472243186433550122 ) ) ;
#1442=DIRECTION ( 'NONE',  ( 0.000000000000000000, -0.9999939076577903929, 0.003490651415223739937 ) ) ;
#1443=EDGE_LOOP ( 'NONE', ( #44686, #21921 ) ) ;
#1444=CARTESIAN_POINT ( 'NONE',  ( 3.349999999999942801, 2.500000000000000000, 2.957883832488649389 ) ) ;
#1446=CARTESIAN_POINT ( 'NONE',  ( 13.74999999999989342, 2.500000000000000000, -1.572243186433550211 ) ) ;
#1447=LINE ( 'NONE', #102858, #84868 ) ;
#1448=CARTESIAN_POINT ( 'NONE',  ( -3.950000000000024603, 2.500000000000000000, -2.411473670974877859 ) ) ;
#1449=DIRECTION ( 'NONE',  ( 0.000000000000000000, 0.000000000000000000, -1.000000000000000000 ) ) ;
#1450=LINE ( 'NONE', #70843, #115246 ) ;
#1451=EDGE_LOOP ( 'NONE', ( #103006, #91378 ) ) ;
#1452=EDGE_LOOP ( 'NONE', ( #64604, #82814 ) ) ;
#1453=CARTESIAN_POINT ( 'NONE',  ( -13.29999999999998828, 2.500000000000000000, 4.430127018922196847 ) ) ;
#1454=ORIENTED_EDGE ( 'NONE', *, *, #49195, .T. ) ;
#1455=LINE ( 'NONE', #100942, #43379 ) ;
#1456=CARTESIAN_POINT ( 'NONE',  ( 2.299999999999949640, 2.500000000000000000, -0.3464101615137782364 ) ) ;
#1457=DIRECTION ( 'NONE',  ( 0.000000000000000000, 1.000000000000000000, 0.000000000000000000 ) ) ;
#1458=ORIENTED_EDGE ( 'NONE', *, *, #2203, .T. ) ;
#1459=EDGE_LOOP ( 'NONE', ( #125884, #66672 ) ) ;
#1460=FACE_BOUND ( 'NONE', #57391, .T. ) ;
#1461=ORIENTED_EDGE ( 'NONE', *, *, #128440, .T. ) ;
#1462=DIRECTION ( 'NONE',  ( 0.000000000000000000, 1.000000000000000000, 0.000000000000000000 ) ) ;
#1463=DIRECTION ( 'NONE',  ( 0.000000000000000000, -0.9999939076577903929, 0.003490651415223739937 ) ) ;
#1464=DIRECTION ( 'NONE',  ( 0.000000000000000000, 1.000000000000000000, 0.000000000000000000 ) ) ;
#1465=CARTESIAN_POINT ( 'NONE',  ( -9.150000000000005684, 2.500000000000000000, 6.595190528383296780 ) ) ;
#1466=CARTESIAN_POINT ( 'NONE',  ( -8.749999999999975131, 12.50000000000000000, 2.099970236277060032 ) ) ;
#1467=CIRCLE ( 'NONE', #124818, 0.1000000000000002554 ) ;
#1468=CARTESIAN_POINT ( 'NONE',  ( 6.849999999999929479, 2.500000000000000000, -2.511473670974877948 ) ) ;
#1469=DIRECTION ( 'NONE',  ( -0.000000000000000000, -1.000000000000000000, -0.000000000000000000 ) ) ;
#1470=CARTESIAN_POINT ( 'NONE',  ( -3.150000000000033218, 12.50000000000000000, -6.841600689897078702 ) ) ;
#1471=CARTESIAN_POINT ( 'NONE',  ( -8.150000000000009237, 12.50000000000000000, 6.083687093685482772 ) ) ;
#1472=LINE ( 'NONE', #21116, #128183 ) ;
#1473=DIRECTION ( 'NONE',  ( 0.000000000000000000, 0.000000000000000000, -1.000000000000000000 ) ) ;
#1474=AXIS2_PLACEMENT_3D ( 'NONE', #28142, #117777, #65470 ) ;
#1475=AXIS2_PLACEMENT_3D ( 'NONE', #13618, #73199, #90902 ) ;
#1476=EDGE_CURVE ( 'NONE', #5550, #44934, #23863, .T. ) ;
#1477=ORIENTED_EDGE ( 'NONE', *, *, #31433, .F. ) ;
#1478=VERTEX_POINT ( 'NONE', #10649 ) ;
#1479=EDGE_LOOP ( 'NONE', ( #86829, #111611, #47767, #112960 ) ) ;
#1480=ORIENTED_EDGE ( 'NONE', *, *, #104369, .F. ) ;
#1481=CARTESIAN_POINT ( 'NONE',  ( -8.300000000000011369, 12.50000000000000000, -4.330127018922201643 ) ) ;
#1482=DIRECTION ( 'NONE',  ( 0.000000000000000000, 0.000000000000000000, -1.000000000000000000 ) ) ;
#1483=ORIENTED_EDGE ( 'NONE', *, *, #1655, .F. ) ;
#1484=ORIENTED_EDGE ( 'NONE', *, *, #47971, .T. ) ;
#1485=ORIENTED_EDGE ( 'NONE', *, *, #41052, .F. ) ;
#1486=CARTESIAN_POINT ( 'NONE',  ( -13.54999999999999005, 2.500000000000000000, -1.918653347947324006 ) ) ;
#1487=CONICAL_SURFACE ( 'NONE', #74645, 0.1000000000000002554, 0.003490658503988666988 ) ;
#1488=AXIS2_PLACEMENT_3D ( 'NONE', #13005, #52966, #92904 ) ;
#1489=AXIS2_PLACEMENT_3D ( 'NONE', #12709, #100466, #89990 ) ;
#1490=DIRECTION ( 'NONE',  ( 0.000000000000000000, 1.000000000000000000, 0.000000000000000000 ) ) ;
#1491=DIRECTION ( 'NONE',  ( 0.000000000000000000, 0.000000000000000000, 1.000000000000000000 ) ) ;
#1492=CARTESIAN_POINT ( 'NONE',  ( -6.250000000000019540, 2.500000000000000000, -2.857883832488653741 ) ) ;
#1493=LINE ( 'NONE', #31616, #118766 ) ;
#1494=EDGE_CURVE ( 'NONE', #126431, #111547, #44793, .T. ) ;
#1495=CARTESIAN_POINT ( 'NONE',  ( 11.64999999999990798, 2.500000000000000000, 7.088010851410848190 ) ) ;
#1496=ADVANCED_FACE ( 'NONE', ( #72828 ), #116493, .T. ) ;
#1497=ORIENTED_EDGE ( 'NONE', *, *, #44549, .T. ) ;
#1498=DIRECTION ( 'NONE',  ( -0.000000000000000000, -1.000000000000000000, -0.000000000000000000 ) ) ;
#1499=ORIENTED_EDGE ( 'NONE', *, *, #101448, .T. ) ;
#1500=VERTEX_POINT ( 'NONE', #81371 ) ;
#1501=VERTEX_POINT ( 'NONE', #122575 ) ;
#1502=DIRECTION ( 'NONE',  ( 0.000000000000000000, 1.000000000000000000, 0.000000000000000000 ) ) ;
#1503=ORIENTED_EDGE ( 'NONE', *, *, #53326, .T. ) ;
#1504=EDGE_CURVE ( 'NONE', #20597, #48724, #112756, .T. ) ;
#1505=EDGE_LOOP ( 'NONE', ( #86966, #46034, #1880, #27546 ) ) ;
#1506=ORIENTED_EDGE ( 'NONE', *, *, #14929, .T. ) ;
#1507=VECTOR ( 'NONE', #92268, 1000.000000000000000 ) ;
#1509=DIRECTION ( 'NONE',  ( -0.000000000000000000, -1.000000000000000000, -0.000000000000000000 ) ) ;
#1510=AXIS2_PLACEMENT_3D ( 'NONE', #129124, #37509, #47321 ) ;
#1511=CARTESIAN_POINT ( 'NONE',  ( -11.84999999999999787, 2.500000000000000000, -6.741600689897073728 ) ) ;
#1512=DIRECTION ( 'NONE',  ( 0.000000000000000000, 0.000000000000000000, 1.000000000000000000 ) ) ;
#1513=DIRECTION ( 'NONE',  ( -0.000000000000000000, -1.000000000000000000, -0.000000000000000000 ) ) ;
#1514=CIRCLE ( 'NONE', #72635, 0.1000000000000002554 ) ;
#1515=FACE_OUTER_BOUND ( 'NONE', #37511, .T. ) ;
#1516=AXIS2_PLACEMENT_3D ( 'NONE', #4333, #11604, #122217 ) ;
#1517=ORIENTED_EDGE ( 'NONE', *, *, #114538, .T. ) ;
#1518=CONICAL_SURFACE ( 'NONE', #26667, 0.1000000000000002554, 0.003490658503988666988 ) ;
#1519=DIRECTION ( 'NONE',  ( 0.000000000000000000, -0.000000000000000000, 1.000000000000000000 ) ) ;
#1520=EDGE_LOOP ( 'NONE', ( #101696, #91460 ) ) ;
#1521=CARTESIAN_POINT ( 'NONE',  ( 7.099999999999928590, 12.50000000000000000, 3.572213422710607489 ) ) ;
#1522=CARTESIAN_POINT ( 'NONE',  ( 0.1999999999999576006, 12.50000000000000000, -4.676537180435978769 ) ) ;
#1523=VERTEX_POINT ( 'NONE', #110178 ) ;
#1524=DIRECTION ( 'NONE',  ( -0.000000000000000000, -1.000000000000000000, -0.000000000000000000 ) ) ;
#1525=VERTEX_POINT ( 'NONE', #861 ) ;
#1526=DIRECTION ( 'NONE',  ( 0.000000000000000000, 0.000000000000000000, 1.000000000000000000 ) ) ;
#1527=EDGE_CURVE ( 'NONE', #13290, #20697, #51764, .T. ) ;
#1528=VECTOR ( 'NONE', #99732, 1000.000000000000000 ) ;
#1529=AXIS2_PLACEMENT_3D ( 'NONE', #46535, #76655, #108037 ) ;
#1530=LINE ( 'NONE', #42115, #88478 ) ;
#1531=EDGE_LOOP ( 'NONE', ( #12078, #21547 ) ) ;
#1532=ORIENTED_EDGE ( 'NONE', *, *, #68147, .T. ) ;
#1533=DIRECTION ( 'NONE',  ( 0.000000000000000000, 0.000000000000000000, -1.000000000000000000 ) ) ;
#1534=CARTESIAN_POINT ( 'NONE',  ( 8.549999999999924327, 2.500000000000000000, 1.718653347947321386 ) ) ;
#1535=EDGE_CURVE ( 'NONE', #118142, #30008, #5758, .T. ) ;
#1537=FACE_OUTER_BOUND ( 'NONE', #100316, .T. ) ;
#1538=EDGE_CURVE ( 'NONE', #39278, #122805, #62234, .T. ) ;
#1539=CARTESIAN_POINT ( 'NONE',  ( -8.350000000000008527, 2.500000000000000000, 5.802370205355744659 ) ) ;
#1540=ORIENTED_EDGE ( 'NONE', *, *, #125339, .T. ) ;
#1541=DIRECTION ( 'NONE',  ( 0.000000000000000000, 0.000000000000000000, 1.000000000000000000 ) ) ;
#1542=EDGE_CURVE ( 'NONE', #54932, #127552, #45513, .T. ) ;
#1543=ADVANCED_FACE ( 'NONE', ( #71524 ), #92454, .T. ) ;
#1544=EDGE_CURVE ( 'NONE', #109083, #54236, #103992, .T. ) ;
#1545=VECTOR ( 'NONE', #55567, 1000.000000000000000 ) ;
#1546=EDGE_CURVE ( 'NONE', #22099, #41508, #14081, .T. ) ;
#1547=EDGE_LOOP ( 'NONE', ( #100115, #18678, #20513, #77162 ) ) ;
#1548=FACE_OUTER_BOUND ( 'NONE', #17091, .T. ) ;
#1549=DIRECTION ( 'NONE',  ( -0.000000000000000000, -1.000000000000000000, -0.000000000000000000 ) ) ;
#1550=EDGE_CURVE ( 'NONE', #29645, #16079, #47561, .T. ) ;
#1552=DIRECTION ( 'NONE',  ( 0.000000000000000000, 0.000000000000000000, 1.000000000000000000 ) ) ;
#1553=DIRECTION ( 'NONE',  ( 0.000000000000000000, 0.000000000000000000, 1.000000000000000000 ) ) ;
#1554=DIRECTION ( 'NONE',  ( 0.000000000000000000, 1.000000000000000000, 0.000000000000000000 ) ) ;
#1555=CARTESIAN_POINT ( 'NONE',  ( 14.14999999999989733, 2.500000000000000000, 1.472243186433545459 ) ) ;
#1556=VERTEX_POINT ( 'NONE', #62373 ) ;
#1557=EDGE_CURVE ( 'NONE', #14107, #20554, #61063, .T. ) ;
#1558=AXIS2_PLACEMENT_3D ( 'NONE', #75074, #73772, #3117 ) ;
#1559=DIRECTION ( 'NONE',  ( -0.000000000000000000, -1.000000000000000000, -0.000000000000000000 ) ) ;
#1560=AXIS2_PLACEMENT_3D ( 'NONE', #83976, #123908, #36197 ) ;
#1561=CARTESIAN_POINT ( 'NONE',  ( -7.500000000000015099, 2.500000000000000000, -0.5928203230275541635 ) ) ;
#1562=DIRECTION ( 'NONE',  ( 0.000000000000000000, 1.000000000000000000, 0.000000000000000000 ) ) ;
#1563=ORIENTED_EDGE ( 'NONE', *, *, #37850, .F. ) ;
#1564=CONICAL_SURFACE ( 'NONE', #112308, 0.09999999999999982514, 0.003490658503988666988 ) ;
#1565=AXIS2_PLACEMENT_3D ( 'NONE', #35225, #114402, #14883 ) ;
#1566=CARTESIAN_POINT ( 'NONE',  ( -4.150000000000027889, 12.50000000000000000, -6.495190528383302464 ) ) ;
#1567=VECTOR ( 'NONE', #124513, 1000.000000000000000 ) ;
#1568=ORIENTED_EDGE ( 'NONE', *, *, #103239, .F. ) ;
#1569=ORIENTED_EDGE ( 'NONE', *, *, #59789, .F. ) ;
#1570=FACE_OUTER_BOUND ( 'NONE', #73684, .T. ) ;
#1571=ORIENTED_EDGE ( 'NONE', *, *, #47825, .T. ) ;
#1572=CARTESIAN_POINT ( 'NONE',  ( 17.84432265422648101, -2.533187527837326591, -5.021315468710856322 ) ) ;
#1573=DIRECTION ( 'NONE',  ( 0.000000000000000000, 0.000000000000000000, 1.000000000000000000 ) ) ;
#1574=AXIS2_PLACEMENT_3D ( 'NONE', #16025, #34421, #5561 ) ;
#1575=ORIENTED_EDGE ( 'NONE', *, *, #38640, .F. ) ;
#1576=AXIS2_PLACEMENT_3D ( 'NONE', #57161, #97090, #7402 ) ;
#1577=CARTESIAN_POINT ( 'NONE',  ( -6.450000000000019718, 2.500000000000000000, -6.148780366869526226 ) ) ;
#1578=CARTESIAN_POINT ( 'NONE',  ( -12.09999999999999609, 12.50000000000000000, -5.022947341949751454 ) ) ;
#1579=EDGE_LOOP ( 'NONE', ( #111478, #116715, #36521, #1047 ) ) ;
#1580=VECTOR ( 'NONE', #61651, 1000.000000000000000 ) ;
#1581=ADVANCED_FACE ( 'NONE', ( #32926 ), #124918, .T. ) ;
#1582=ORIENTED_EDGE ( 'NONE', *, *, #116388, .F. ) ;
#1583=EDGE_LOOP ( 'NONE', ( #10309, #54978, #30149, #12881 ) ) ;
#1584=DIRECTION ( 'NONE',  ( 0.000000000000000000, 1.000000000000000000, 0.000000000000000000 ) ) ;
#1585=CARTESIAN_POINT ( 'NONE',  ( -3.100000000000028511, 2.500000000000000000, -3.883716857408426648 ) ) ;
#1586=CARTESIAN_POINT ( 'NONE',  ( 11.89999999999990443, 12.50000000000000000, -0.2813168883297408329 ) ) ;
#1587=FACE_BOUND ( 'NONE', #51323, .T. ) ;
#1588=EDGE_LOOP ( 'NONE', ( #64511, #122818 ) ) ;
#1589=VECTOR ( 'NONE', #37866, 1000.000000000000000 ) ;
#1590=DIRECTION ( 'NONE',  ( -0.000000000000000000, 1.000000000000000000, -0.000000000000000000 ) ) ;
#1591=DIRECTION ( 'NONE',  ( -0.000000000000000000, -1.000000000000000000, -0.000000000000000000 ) ) ;
#1592=AXIS2_PLACEMENT_3D ( 'NONE', #107180, #7685, #89484 ) ;
#1593=ORIENTED_EDGE ( 'NONE', *, *, #83190, .F. ) ;
#1594=EDGE_CURVE ( 'NONE', #122488, #118638, #63003, .T. ) ;
#1595=CARTESIAN_POINT ( 'NONE',  ( -10.80000000000000249, 2.500000000000000000, -4.330127018922197202 ) ) ;
#1596=PLANE ( 'NONE',  #9499 ) ;
#1597=AXIS2_PLACEMENT_3D ( 'NONE', #6212, #114251, #85435 ) ;
#1598=CARTESIAN_POINT ( 'NONE',  ( 9.349999999999916156, 2.500000000000000000, 6.148780366869520009 ) ) ;
#1599=LINE ( 'NONE', #84023, #42958 ) ;
#1600=CARTESIAN_POINT ( 'NONE',  ( -9.600000000000006750, 12.50000000000000000, -0.6277270498435167934 ) ) ;
#1601=LINE ( 'NONE', #110277, #88988 ) ;
#1602=VECTOR ( 'NONE', #125277, 1000.000000000000000 ) ;
#1603=FACE_OUTER_BOUND ( 'NONE', #60406, .T. ) ;
#1604=AXIS2_PLACEMENT_3D ( 'NONE', #112241, #63791, #103716 ) ;
#1605=CIRCLE ( 'NONE', #43490, 0.06509327318403745899 ) ;
#1606=ORIENTED_EDGE ( 'NONE', *, *, #4797, .T. ) ;
#1607=ORIENTED_EDGE ( 'NONE', *, *, #89892, .T. ) ;
#1608=ORIENTED_EDGE ( 'NONE', *, *, #108778, .F. ) ;
#1609=VERTEX_POINT ( 'NONE', #93120 ) ;
#1610=LINE ( 'NONE', #90645, #91377 ) ;
#1611=CARTESIAN_POINT ( 'NONE',  ( 12.69999999999990337, 2.500000000000000000, 3.983716857408420076 ) ) ;
#1612=VECTOR ( 'NONE', #128044, 1000.000000000000000 ) ;
#1613=ORIENTED_EDGE ( 'NONE', *, *, #16015, .T. ) ;
#1614=FACE_BOUND ( 'NONE', #122207, .T. ) ;
#1615=CARTESIAN_POINT ( 'NONE',  ( -10.60000000000000320, 12.50000000000000000, -3.983716857408421852 ) ) ;
#1616=CARTESIAN_POINT ( 'NONE',  ( 1.049999999999953637, 12.50000000000000000, -1.818653347947326138 ) ) ;
#1620=CARTESIAN_POINT ( 'NONE',  ( -4.550000000000022915, 2.500000000000000000, 2.165063509461097713 ) ) ;
#1621=CARTESIAN_POINT ( 'NONE',  ( -8.100000000000013856, 2.500000000000000000, -0.3464101615137782364 ) ) ;
#1622=CARTESIAN_POINT ( 'NONE',  ( 7.699999999999922018, 2.500000000000000000, 0.3464101615137735735 ) ) ;
#1623=( BOUNDED_SURFACE ( )  B_SPLINE_SURFACE ( 2, 3, ( 
 ( #37303, #126319, #127607, #77848 ),
 ( #77220, #117759, #88972, #57590 ),
 ( #28117, #56277, #107966, #128268 ),
 ( #47125, #88302, #96194, #6499 ),
 ( #26830, #86382, #58865, #9118 ) ),
 .UNSPECIFIED., .F., .F., .F. ) 
 B_SPLINE_SURFACE_WITH_KNOTS ( ( 3, 2, 3 ),
 ( 4, 4 ),
 ( 0.000000000000000000, 1.000000000000000000, 1.133771318130139871 ),
 ( -0.0002500000000000000052, 0.005250000000000000326 ),
 .UNSPECIFIED. ) 
 GEOMETRIC_REPRESENTATION_ITEM ( )  RATIONAL_B_SPLINE_SURFACE ( (
 ( 1.000000000000000000, 1.000000000000000000, 1.000000000000000000, 1.000000000000000000),
 ( 0.7071067811865475727, 0.7071067811865475727, 0.7071067811865475727, 0.7071067811865475727),
 ( 1.000000000000000000, 1.000000000000000000, 1.000000000000000000, 1.000000000000000000),
 ( 1.000000000000000000, 1.000000000000000000, 1.000000000000000000, 1.000000000000000000),
 ( 1.000000000000000000, 1.000000000000000000, 1.000000000000000000, 1.000000000000000000) ) ) 
 REPRESENTATION_ITEM ( '' )  SURFACE ( )  );
#1624=CARTESIAN_POINT ( 'NONE',  ( -2.950000000000030376, 2.500000000000000000, 6.495190528383297135 ) ) ;
#1625=CARTESIAN_POINT ( 'NONE',  ( -1.450000000000035039, 12.50000000000000000, -6.841600689897077814 ) ) ;
#1626=CARTESIAN_POINT ( 'NONE',  ( -0.4000000000000339950, 2.500000000000000000, 0.7928203230275517877 ) ) ;
#1627=ORIENTED_EDGE ( 'NONE', *, *, #19572, .F. ) ;
#1628=EDGE_LOOP ( 'NONE', ( #87048, #126957, #21833, #6855 ) ) ;
#1631=ORIENTED_EDGE ( 'NONE', *, *, #14352, .T. ) ;
#1632=ORIENTED_EDGE ( 'NONE', *, *, #12805, .F. ) ;
#1633=ORIENTED_EDGE ( 'NONE', *, *, #80465, .F. ) ;
#1634=ORIENTED_EDGE ( 'NONE', *, *, #126096, .F. ) ;
#1635=DIRECTION ( 'NONE',  ( 0.000000000000000000, 1.000000000000000000, 0.000000000000000000 ) ) ;
#1636=ORIENTED_EDGE ( 'NONE', *, *, #31142, .F. ) ;
#1637=EDGE_CURVE ( 'NONE', #74213, #62109, #45309, .T. ) ;
#1638=DIRECTION ( 'NONE',  ( 0.000000000000000000, 0.000000000000000000, 1.000000000000000000 ) ) ;
#1639=DIRECTION ( 'NONE',  ( -0.000000000000000000, 1.000000000000000000, -0.000000000000000000 ) ) ;
#1640=CARTESIAN_POINT ( 'NONE',  ( 2.099999999999949463, 2.500000000000000000, -3.637306695894650055 ) ) ;
#1641=DIRECTION ( 'NONE',  ( 0.000000000000000000, 0.000000000000000000, -1.000000000000000000 ) ) ;
#1642=CIRCLE ( 'NONE', #129227, 0.06509327318403743123 ) ;
#1643=ADVANCED_FACE ( 'NONE', ( #54464 ), #122771, .T. ) ;
#1644=ADVANCED_FACE ( 'NONE', ( #105512 ), #87241, .T. ) ;
#1645=VERTEX_POINT ( 'NONE', #4694 ) ;
#1646=CARTESIAN_POINT ( 'NONE',  ( -6.450000000000019718, 2.500000000000000000, -1.818653347947326138 ) ) ;
#1647=CONICAL_SURFACE ( 'NONE', #85278, 0.1000000000000002554, 0.003490658503988666988 ) ;
#1648=EDGE_LOOP ( 'NONE', ( #39907, #129114, #125910, #101323 ) ) ;
#1649=AXIS2_PLACEMENT_3D ( 'NONE', #79969, #87202, #98968 ) ;
#1650=ORIENTED_EDGE ( 'NONE', *, *, #89470, .F. ) ;
#1651=DIRECTION ( 'NONE',  ( -0.000000000000000000, -1.000000000000000000, -0.000000000000000000 ) ) ;
#1652=EDGE_CURVE ( 'NONE', #36694, #85926, #95692, .T. ) ;
#1653=CARTESIAN_POINT ( 'NONE',  ( -12.89999999999999147, 12.50000000000000000, 4.330127018922196314 ) ) ;
#1654=DIRECTION ( 'NONE',  ( -0.000000000000000000, 1.000000000000000000, -0.000000000000000000 ) ) ;
#1655=EDGE_CURVE ( 'NONE', #124666, #40568, #58027, .T. ) ;
#1656=EDGE_LOOP ( 'NONE', ( #124418, #42763 ) ) ;
#1657=AXIS2_PLACEMENT_3D ( 'NONE', #58736, #98635, #88830 ) ;
#1659=CARTESIAN_POINT ( 'NONE',  ( 0.8499999999999553468, 12.50000000000000000, -2.165063509461101710 ) ) ;
#1660=DIRECTION ( 'NONE',  ( -0.000000000000000000, 1.000000000000000000, -0.000000000000000000 ) ) ;
#1661=DIRECTION ( 'NONE',  ( 0.000000000000000000, 0.000000000000000000, 1.000000000000000000 ) ) ;
#1662=CARTESIAN_POINT ( 'NONE',  ( 8.349999999999919709, 12.50000000000000000, -1.407149913249512663 ) ) ;
#1664=DIRECTION ( 'NONE',  ( 0.000000000000000000, 0.000000000000000000, -1.000000000000000000 ) ) ;
#1665=ORIENTED_EDGE ( 'NONE', *, *, #99190, .F. ) ;
#1666=CARTESIAN_POINT ( 'NONE',  ( 14.93723468728801507, -2.499999999999999112, 6.174425104148753896 ) ) ;
#1667=AXIS2_PLACEMENT_3D ( 'NONE', #84534, #74072, #104798 ) ;
#1668=ORIENTED_EDGE ( 'NONE', *, *, #111949, .T. ) ;
#1669=DIRECTION ( 'NONE',  ( -0.000000000000000000, -1.000000000000000000, -0.000000000000000000 ) ) ;
#1670=DIRECTION ( 'NONE',  ( 0.000000000000000000, -0.9999939076577903929, 0.003490651415223739937 ) ) ;
#1671=CARTESIAN_POINT ( 'NONE',  ( -8.749999999999975131, 2.500000000000000000, 2.265063509461097357 ) ) ;
#1672=AXIS2_PLACEMENT_3D ( 'NONE', #78183, #118088, #59192 ) ;
#1673=DIRECTION ( 'NONE',  ( 0.000000000000000000, 1.000000000000000000, 0.000000000000000000 ) ) ;
#1674=DIRECTION ( 'NONE',  ( 0.000000000000000000, 0.000000000000000000, 1.000000000000000000 ) ) ;
#1675=ORIENTED_EDGE ( 'NONE', *, *, #80020, .T. ) ;
#1676=DIRECTION ( 'NONE',  ( -0.000000000000000000, 1.000000000000000000, -0.000000000000000000 ) ) ;
#1677=AXIS2_PLACEMENT_3D ( 'NONE', #116368, #37191, #26716 ) ;
#1679=PLANE ( 'NONE',  #46523 ) ;
#1680=EDGE_LOOP ( 'NONE', ( #122884, #69929 ) ) ;
#1681=ORIENTED_EDGE ( 'NONE', *, *, #117977, .F. ) ;
#1682=EDGE_LOOP ( 'NONE', ( #119202, #20973, #82004, #126348 ) ) ;
#1683=CARTESIAN_POINT ( 'NONE',  ( 17.50000000000000000, -0.9166666666666696273, 2.864912725862981624 ) ) ;
#1684=DIRECTION ( 'NONE',  ( -0.000000000000000000, -1.000000000000000000, -0.000000000000000000 ) ) ;
#1687=CARTESIAN_POINT ( 'NONE',  ( -8.750000000000008882, 2.500000000000000000, -2.957883832488653830 ) ) ;
#1688=CIRCLE ( 'NONE', #7950, 0.1000000000000002554 ) ;
#1689=CARTESIAN_POINT ( 'NONE',  ( -3.642919299551294898E-14, 2.500000000000000000, 0.7928203230275517877 ) ) ;
#1690=EDGE_CURVE ( 'NONE', #55973, #54643, #125147, .T. ) ;
#1691=CARTESIAN_POINT ( 'NONE',  ( -11.69999999999999929, 2.500000000000000000, -4.430127018922199511 ) ) ;
#1692=DIRECTION ( 'NONE',  ( 0.000000000000000000, 0.000000000000000000, -1.000000000000000000 ) ) ;
#1693=CARTESIAN_POINT ( 'NONE',  ( 8.349999999999923261, 12.50000000000000000, 1.537336459617582918 ) ) ;
#1694=EDGE_CURVE ( 'NONE', #129065, #13310, #26621, .T. ) ;
#1695=EDGE_CURVE ( 'NONE', #119558, #2346, #9897, .T. ) ;
#1696=AXIS2_PLACEMENT_3D ( 'NONE', #73430, #112734, #94360 ) ;
#1697=EDGE_CURVE ( 'NONE', #68225, #38667, #93754, .T. ) ;
#1699=EDGE_LOOP ( 'NONE', ( #70879, #8956 ) ) ;
#1700=EDGE_CURVE ( 'NONE', #92524, #46914, #3635, .T. ) ;
#1701=DIRECTION ( 'NONE',  ( -0.000000000000000000, 1.000000000000000000, -0.000000000000000000 ) ) ;
#1702=VECTOR ( 'NONE', #67936, 1000.000000000000000 ) ;
#1703=DIRECTION ( 'NONE',  ( 0.000000000000000000, 0.000000000000000000, 1.000000000000000000 ) ) ;
#1704=DIRECTION ( 'NONE',  ( 0.000000000000000000, 0.000000000000000000, -1.000000000000000000 ) ) ;
#1705=CARTESIAN_POINT ( 'NONE',  ( -11.84999999999999787, 12.50000000000000000, -2.511473670974873951 ) ) ;
#1706=ORIENTED_EDGE ( 'NONE', *, *, #57819, .F. ) ;
#1707=ADVANCED_FACE ( 'NONE', ( #4071 ), #49719, .T. ) ;
#1708=CARTESIAN_POINT ( 'NONE',  ( -8.350000000000013856, 2.500000000000000000, -5.702370205355745014 ) ) ;
#1709=CIRCLE ( 'NONE', #22666, 0.06509327318403745899 ) ;
#1710=AXIS2_PLACEMENT_3D ( 'NONE', #52444, #93668, #4603 ) ;
#1711=ADVANCED_FACE ( 'NONE', ( #44019 ), #106040, .T. ) ;
#1712=CARTESIAN_POINT ( 'NONE',  ( 13.29999999999990301, 2.500000000000000000, 4.230127018922196669 ) ) ;
#1713=CARTESIAN_POINT ( 'NONE',  ( 13.54999999999989946, 2.500000000000000000, 2.411473670974873862 ) ) ;
#1714=ORIENTED_EDGE ( 'NONE', *, *, #69909, .F. ) ;
#1715=EDGE_LOOP ( 'NONE', ( #99532, #98552, #53633, #123665 ) ) ;
#1716=DIRECTION ( 'NONE',  ( -0.000000000000000000, -1.000000000000000000, -0.000000000000000000 ) ) ;
#1717=EDGE_LOOP ( 'NONE', ( #7917, #95060 ) ) ;
#1718=ORIENTED_EDGE ( 'NONE', *, *, #67888, .T. ) ;
#1719=CARTESIAN_POINT ( 'NONE',  ( -10.80000000000000071, 2.500000000000000000, 4.230127018922196669 ) ) ;
#1720=VECTOR ( 'NONE', #87234, 1000.000000000000000 ) ;
#1721=ADVANCED_FACE ( 'NONE', ( #73456 ), #65573, .T. ) ;
#1722=CARTESIAN_POINT ( 'NONE',  ( 20.64614705759136015, 2.669560853936051803, -2.247897417617913618 ) ) ;
#1723=FACE_OUTER_BOUND ( 'NONE', #80418, .T. ) ;
#1724=DIRECTION ( 'NONE',  ( 0.000000000000000000, 1.000000000000000000, 0.000000000000000000 ) ) ;
#1725=VERTEX_POINT ( 'NONE', #125763 ) ;
#1726=CIRCLE ( 'NONE', #116747, 0.1000000000000002554 ) ;
#1727=VECTOR ( 'NONE', #90995, 1000.000000000000000 ) ;
#1728=AXIS2_PLACEMENT_3D ( 'NONE', #37888, #80405, #128217 ) ;
#1729=FACE_OUTER_BOUND ( 'NONE', #112827, .T. ) ;
#1730=VERTEX_POINT ( 'NONE', #36125 ) ;
#1731=CARTESIAN_POINT ( 'NONE',  ( -2.050000000000033129, 12.50000000000000000, 2.230156782645134950 ) ) ;
#1732=DIRECTION ( 'NONE',  ( 0.000000000000000000, 1.000000000000000000, 0.000000000000000000 ) ) ;
#1733=VERTEX_POINT ( 'NONE', #24369 ) ;
#1734=CONICAL_SURFACE ( 'NONE', #10164, 0.1000000000000002554, 0.003490658503988666988 ) ;
#1735=AXIS2_PLACEMENT_3D ( 'NONE', #124187, #66542, #114358 ) ;
#1736=ORIENTED_EDGE ( 'NONE', *, *, #62762, .F. ) ;
#1738=VERTEX_POINT ( 'NONE', #26310 ) ;
#1739=LINE ( 'NONE', #90113, #23146 ) ;
#1740=CARTESIAN_POINT ( 'NONE',  ( 15.22989033368257950, 2.499999999999486633, 7.180069491320466568 ) ) ;
#1741=DIRECTION ( 'NONE',  ( 0.000000000000000000, 1.000000000000000000, 0.000000000000000000 ) ) ;
#1742=FACE_BOUND ( 'NONE', #81437, .T. ) ;
#1743=ORIENTED_EDGE ( 'NONE', *, *, #72468, .F. ) ;
#1744=CARTESIAN_POINT ( 'NONE',  ( -12.29999999999999538, 2.500000000000000000, -4.676537180435976104 ) ) ;
#1746=CIRCLE ( 'NONE', #85383, 0.06509327318403745899 ) ;
#1747=CARTESIAN_POINT ( 'NONE',  ( 13.14999999999990088, 2.500000000000000000, 2.511473670974873507 ) ) ;
#1748=CARTESIAN_POINT ( 'NONE',  ( 1.049999999999954969, 2.500000000000000000, -6.941600689897077459 ) ) ;
#1749=EDGE_CURVE ( 'NONE', #29970, #98422, #85199, .T. ) ;
#1750=AXIS2_PLACEMENT_3D ( 'NONE', #14406, #116475, #75914 ) ;
#1751=CARTESIAN_POINT ( 'NONE',  ( -3.750000000000025757, 12.50000000000000000, 1.472243186433545459 ) ) ;
#1752=FACE_OUTER_BOUND ( 'NONE', #45837, .T. ) ;
#1753=FACE_OUTER_BOUND ( 'NONE', #56528, .T. ) ;
#1754=AXIS2_PLACEMENT_3D ( 'NONE', #92929, #123026, #44456 ) ;
#1755=DIRECTION ( 'NONE',  ( 0.000000000000000000, 1.000000000000000000, 0.000000000000000000 ) ) ;
#1756=EDGE_LOOP ( 'NONE', ( #44364, #81307 ) ) ;
#1757=VERTEX_POINT ( 'NONE', #14525 ) ;
#1758=EDGE_LOOP ( 'NONE', ( #81359, #118787, #83378, #9902 ) ) ;
#1759=ORIENTED_EDGE ( 'NONE', *, *, #85925, .F. ) ;
#1760=VERTEX_POINT ( 'NONE', #23732 ) ;
#1761=VECTOR ( 'NONE', #57075, 1000.000000000000000 ) ;
#1762=CARTESIAN_POINT ( 'NONE',  ( -14.39999999999998614, 2.500000000000000000, -0.2464101615137760659 ) ) ;
#1763=CARTESIAN_POINT ( 'NONE',  ( -13.54999999999998828, 12.50000000000000000, 1.818653347947325472 ) ) ;
#1765=FACE_BOUND ( 'NONE', #79748, .T. ) ;
#1766=CARTESIAN_POINT ( 'NONE',  ( -3.550000000000027356, 2.500000000000000000, -2.411473670974877859 ) ) ;
#1767=AXIS2_PLACEMENT_3D ( 'NONE', #111146, #61445, #101361 ) ;
#1768=ORIENTED_EDGE ( 'NONE', *, *, #14795, .F. ) ;
#1769=DIRECTION ( 'NONE',  ( 0.000000000000000000, 0.000000000000000000, 1.000000000000000000 ) ) ;
#1770=DIRECTION ( 'NONE',  ( 0.000000000000000000, 0.000000000000000000, -1.000000000000000000 ) ) ;
#1771=FACE_OUTER_BOUND ( 'NONE', #67507, .T. ) ;
#1772=CARTESIAN_POINT ( 'NONE',  ( -1.900000000000034550, 2.500000000000000000, 4.676537180435972552 ) ) ;
#1773=EDGE_LOOP ( 'NONE', ( #63223, #58049, #57994, #59182 ) ) ;
#1774=CIRCLE ( 'NONE', #72812, 0.06509327318403745899 ) ;
#1775=FACE_OUTER_BOUND ( 'NONE', #66052, .T. ) ;
#1776=VERTEX_POINT ( 'NONE', #113382 ) ;
#1777=EDGE_LOOP ( 'NONE', ( #30067, #66294, #114054, #128798 ) ) ;
#1778=DIRECTION ( 'NONE',  ( 0.000000000000000000, 1.000000000000000000, 0.000000000000000000 ) ) ;
#1779=CARTESIAN_POINT ( 'NONE',  ( -7.700000000000014388, 2.500000000000000000, -4.576537180435977348 ) ) ;
#1780=AXIS2_PLACEMENT_3D ( 'NONE', #75355, #96278, #24978 ) ;
#1781=EDGE_LOOP ( 'NONE', ( #12829, #105421 ) ) ;
#1782=DIRECTION ( 'NONE',  ( 0.000000000000000000, 0.000000000000000000, 1.000000000000000000 ) ) ;
#1784=CARTESIAN_POINT ( 'NONE',  ( 6.049999999999934097, 12.50000000000000000, -2.576566944158915184 ) ) ;
#1785=CARTESIAN_POINT ( 'NONE',  ( -10.45000000000000107, 2.500000000000000000, 2.165063509461097713 ) ) ;
#1786=DIRECTION ( 'NONE',  ( 0.000000000000000000, 0.000000000000000000, -1.000000000000000000 ) ) ;
#1787=CARTESIAN_POINT ( 'NONE',  ( -10.65000000000000391, 2.500000000000000000, -6.941600689897075682 ) ) ;
#1788=VERTEX_POINT ( 'NONE', #17753 ) ;
#1789=AXIS2_PLACEMENT_3D ( 'NONE', #105785, #58630, #46212 ) ;
#1790=ADVANCED_FACE ( 'NONE', ( #99565 ), #109366, .T. ) ;
#1791=FACE_OUTER_BOUND ( 'NONE', #48669, .T. ) ;
#1792=EDGE_CURVE ( 'NONE', #118832, #51819, #89409, .T. ) ;
#1793=ORIENTED_EDGE ( 'NONE', *, *, #105090, .T. ) ;
#1794=FACE_OUTER_BOUND ( 'NONE', #102906, .T. ) ;
#1795=CIRCLE ( 'NONE', #18534, 0.06509327318403745899 ) ;
#1796=AXIS2_PLACEMENT_3D ( 'NONE', #33307, #73216, #83679 ) ;
#1797=ORIENTED_EDGE ( 'NONE', *, *, #33724, .F. ) ;
#1798=DIRECTION ( 'NONE',  ( -0.000000000000000000, -1.000000000000000000, -0.000000000000000000 ) ) ;
#1799=EDGE_LOOP ( 'NONE', ( #33142, #114576, #21469, #104478 ) ) ;
#1800=CARTESIAN_POINT ( 'NONE',  ( -10.60000000000000142, 12.50000000000000000, 4.741630453620009789 ) ) ;
#1801=FACE_OUTER_BOUND ( 'NONE', #20259, .T. ) ;
#1802=EDGE_CURVE ( 'NONE', #54180, #54197, #83071, .T. ) ;
#1803=EDGE_CURVE ( 'NONE', #83051, #56486, #37096, .T. ) ;
#1804=DIRECTION ( 'NONE',  ( 0.000000000000000000, 1.000000000000000000, 0.000000000000000000 ) ) ;
#1805=EDGE_CURVE ( 'NONE', #101014, #844, #53807, .T. ) ;
#1806=DIRECTION ( 'NONE',  ( 0.000000000000000000, -0.9999939076577903929, 0.003490651415223739937 ) ) ;
#1807=ADVANCED_FACE ( 'NONE', ( #127715 ), #14171, .T. ) ;
#1808=CARTESIAN_POINT ( 'NONE',  ( 11.24999999999994493, 12.50000000000000000, 6.495190528383297135 ) ) ;
#1809=ORIENTED_EDGE ( 'NONE', *, *, #114284, .F. ) ;
#1810=ORIENTED_EDGE ( 'NONE', *, *, #2599, .F. ) ;
#1812=DIRECTION ( 'NONE',  ( 0.000000000000000000, 0.000000000000000000, -1.000000000000000000 ) ) ;
#1813=DIRECTION ( 'NONE',  ( 0.000000000000000000, 0.000000000000000000, -1.000000000000000000 ) ) ;
#1814=CARTESIAN_POINT ( 'NONE',  ( -3.550000000000027356, 12.50000000000000000, -2.576566944158915184 ) ) ;
#1815=AXIS2_PLACEMENT_3D ( 'NONE', #38514, #27358, #107869 ) ;
#1816=ORIENTED_EDGE ( 'NONE', *, *, #52997, .F. ) ;
#1817=ORIENTED_EDGE ( 'NONE', *, *, #121797, .F. ) ;
#1818=EDGE_LOOP ( 'NONE', ( #77084, #103594, #92488, #80314 ) ) ;
#1820=DIRECTION ( 'NONE',  ( 0.000000000000000000, 0.000000000000000000, 1.000000000000000000 ) ) ;
#1821=ORIENTED_EDGE ( 'NONE', *, *, #128507, .F. ) ;
#1822=CARTESIAN_POINT ( 'NONE',  ( -9.350000000000008527, 12.50000000000000000, -6.776507416713035248 ) ) ;
#1823=DIRECTION ( 'NONE',  ( -0.000000000000000000, 1.000000000000000000, -0.000000000000000000 ) ) ;
#1824=AXIS2_PLACEMENT_3D ( 'NONE', #98141, #100092, #38610 ) ;
#1825=AXIS2_PLACEMENT_3D ( 'NONE', #10072, #109562, #128584 ) ;
#1826=DIRECTION ( 'NONE',  ( -0.000000000000000000, 1.000000000000000000, -0.000000000000000000 ) ) ;
#1827=LINE ( 'NONE', #19541, #104599 ) ;
#1828=AXIS2_PLACEMENT_3D ( 'NONE', #23389, #53520, #13569 ) ;
#1829=DIRECTION ( 'NONE',  ( 0.000000000000000000, -0.9999939076577903929, 0.003490651415223739937 ) ) ;
#1830=FACE_OUTER_BOUND ( 'NONE', #82276, .T. ) ;
#1831=CARTESIAN_POINT ( 'NONE',  ( -10.00000000000000355, 2.500000000000000000, -0.7928203230275542301 ) ) ;
#1832=FACE_OUTER_BOUND ( 'NONE', #114504, .T. ) ;
#1833=VECTOR ( 'NONE', #105501, 1000.000000000000000 ) ;
#1834=ORIENTED_EDGE ( 'NONE', *, *, #103239, .T. ) ;
#1835=CONICAL_SURFACE ( 'NONE', #106387, 0.09999999999999999167, 0.003490658503988666988 ) ;
#1836=VECTOR ( 'NONE', #90045, 1000.000000000000000 ) ;
#1837=PLANE ( 'NONE',  #36128 ) ;
#1838=CARTESIAN_POINT ( 'NONE',  ( 34.93074629416160803, -2.900242961800562291, 4.640733549227246790 ) ) ;
#1839=EDGE_LOOP ( 'NONE', ( #128772, #75940 ) ) ;
#1842=FACE_OUTER_BOUND ( 'NONE', #82318, .T. ) ;
#1843=CARTESIAN_POINT ( 'NONE',  ( -2.500000000000030642, 2.500000000000000000, -0.7928203230275542301 ) ) ;
#1844=AXIS2_PLACEMENT_3D ( 'NONE', #18655, #118793, #59252 ) ;
#1845=DIRECTION ( 'NONE',  ( 0.000000000000000000, 0.000000000000000000, 1.000000000000000000 ) ) ;
#1846=DIRECTION ( 'NONE',  ( -4.274815082592931898E-19, -0.9999939076577903929, -0.003490651415223739937 ) ) ;
#1847=DIRECTION ( 'NONE',  ( 0.000000000000000000, 0.000000000000000000, -1.000000000000000000 ) ) ;
#1848=CARTESIAN_POINT ( 'NONE',  ( -6.250000000000017764, 2.500000000000000000, 7.188010851410848723 ) ) ;
#1849=DIRECTION ( 'NONE',  ( 0.000000000000000000, -0.9999939076577903929, 0.003490651415223739937 ) ) ;
#1850=EDGE_CURVE ( 'NONE', #55993, #39292, #57031, .T. ) ;
#1851=ADVANCED_FACE ( 'NONE', ( #96964 ), #7287, .T. ) ;
#1852=DIRECTION ( 'NONE',  ( 0.000000000000000000, 0.000000000000000000, 1.000000000000000000 ) ) ;
#1853=VERTEX_POINT ( 'NONE', #28239 ) ;
#1854=ORIENTED_EDGE ( 'NONE', *, *, #97187, .T. ) ;
#1855=ADVANCED_FACE ( 'NONE', ( #7934 ), #43454, .T. ) ;
#1856=ORIENTED_EDGE ( 'NONE', *, *, #13373, .F. ) ;
#1857=CIRCLE ( 'NONE', #35332, 0.06509327318403745899 ) ;
#1858=ORIENTED_EDGE ( 'NONE', *, *, #51957, .T. ) ;
#1859=ADVANCED_FACE ( 'NONE', ( #77970 ), #8568, .T. ) ;
#1860=DIRECTION ( 'NONE',  ( 0.000000000000000000, 0.000000000000000000, -1.000000000000000000 ) ) ;
#1862=EDGE_CURVE ( 'NONE', #97069, #24036, #116601, .T. ) ;
#1863=VERTEX_POINT ( 'NONE', #28888 ) ;
#1864=EDGE_CURVE ( 'NONE', #54180, #45787, #68800, .T. ) ;
#1866=FACE_OUTER_BOUND ( 'NONE', #20948, .T. ) ;
#1867=EDGE_CURVE ( 'NONE', #79959, #108868, #98899, .T. ) ;
#1868=VECTOR ( 'NONE', #100532, 1000.000000000000000 ) ;
#1869=CARTESIAN_POINT ( 'NONE',  ( 12.69999999999990337, 2.500000000000000000, 3.883716857408420431 ) ) ;
#1870=DIRECTION ( 'NONE',  ( -4.274815082592931898E-19, -0.9999939076577903929, -0.003490651415223739937 ) ) ;
#1871=EDGE_LOOP ( 'NONE', ( #54821, #36111 ) ) ;
#1872=DIRECTION ( 'NONE',  ( 0.000000000000000000, -0.9999939076577903929, 0.003490651415223739937 ) ) ;
#1873=VECTOR ( 'NONE', #114832, 1000.000000000000000 ) ;
#1874=ADVANCED_FACE ( 'NONE', ( #89092 ), #9986, .T. ) ;
#1875=DIRECTION ( 'NONE',  ( 0.000000000000000000, 1.000000000000000000, 0.000000000000000000 ) ) ;
#1876=ORIENTED_EDGE ( 'NONE', *, *, #111837, .F. ) ;
#1877=AXIS2_PLACEMENT_3D ( 'NONE', #47145, #7843, #37961 ) ;
#1878=ORIENTED_EDGE ( 'NONE', *, *, #68368, .F. ) ;
#1879=ORIENTED_EDGE ( 'NONE', *, *, #103961, .T. ) ;
#1880=ORIENTED_EDGE ( 'NONE', *, *, #12323, .T. ) ;
#1881=CARTESIAN_POINT ( 'NONE',  ( -9.400000000000007461, 2.500000000000000000, 4.676537180435972552 ) ) ;
#1882=CIRCLE ( 'NONE', #43681, 0.06509327318403741736 ) ;
#1883=CARTESIAN_POINT ( 'NONE',  ( -0.8000000000000381251, 12.50000000000000000, 4.330127018922196314 ) ) ;
#1884=CARTESIAN_POINT ( 'NONE',  ( 8.299999999999922551, 12.50000000000000000, -2.385244779468109755E-15 ) ) ;
#1885=ORIENTED_EDGE ( 'NONE', *, *, #34709, .T. ) ;
#1886=VECTOR ( 'NONE', #79946, 1000.000000000000000 ) ;
#1887=VECTOR ( 'NONE', #113154, 1000.000000000000000 ) ;
#1888=CARTESIAN_POINT ( 'NONE',  ( 10.44999999999991047, 12.50000000000000000, 2.165063509461097713 ) ) ;
#1890=LINE ( 'NONE', #52294, #110239 ) ;
#1891=CARTESIAN_POINT ( 'NONE',  ( 6.649999999999931966, 2.500000000000000000, -7.188010851410854052 ) ) ;
#1892=CONICAL_SURFACE ( 'NONE', #75062, 0.1000000000000002554, 0.003490658503988666988 ) ;
#1893=FACE_OUTER_BOUND ( 'NONE', #63778, .T. ) ;
#1894=CARTESIAN_POINT ( 'NONE',  ( 21.15177371151418839, -2.593223176056364210, 4.151029080743465549 ) ) ;
#1895=ADVANCED_FACE ( 'NONE', ( #41292 ), #60181, .T. ) ;
#1896=ORIENTED_EDGE ( 'NONE', *, *, #27117, .T. ) ;
#1897=CIRCLE ( 'NONE', #102263, 0.09999999999999982514 ) ;
#1898=CIRCLE ( 'NONE', #116905, 0.1000000000000002554 ) ;
#1899=VERTEX_POINT ( 'NONE', #81209 ) ;
#1900=VERTEX_POINT ( 'NONE', #52 ) ;
#1901=DIRECTION ( 'NONE',  ( -4.274815082592931898E-19, -0.9999939076577903929, -0.003490651415223739937 ) ) ;
#1902=DIRECTION ( 'NONE',  ( 0.000000000000000000, 0.000000000000000000, 1.000000000000000000 ) ) ;
#1903=FACE_BOUND ( 'NONE', #74197, .T. ) ;
#1904=DIRECTION ( 'NONE',  ( -0.000000000000000000, -1.000000000000000000, -0.000000000000000000 ) ) ;
#1905=LINE ( 'NONE', #43796, #79948 ) ;
#1906=LINE ( 'NONE', #41223, #91776 ) ;
#1907=EDGE_CURVE ( 'NONE', #93919, #96281, #3719, .T. ) ;
#1908=CARTESIAN_POINT ( 'NONE',  ( 0.8499999999999557909, 12.50000000000000000, -6.495190528383302464 ) ) ;
#1909=DIRECTION ( 'NONE',  ( 0.000000000000000000, -0.9999939076577903929, 0.003490651415223739937 ) ) ;
#1910=CARTESIAN_POINT ( 'NONE',  ( -11.25000000000000000, 12.50000000000000000, 7.188010851410848723 ) ) ;
#1911=ORIENTED_EDGE ( 'NONE', *, *, #8933, .T. ) ;
#1912=CARTESIAN_POINT ( 'NONE',  ( -13.94999999999998685, 2.500000000000000000, 1.818653347947325472 ) ) ;
#1913=CONICAL_SURFACE ( 'NONE', #73026, 0.1000000000000000472, 0.003490658503988666988 ) ;
#1914=CONICAL_SURFACE ( 'NONE', #68823, 0.1000000000000000472, 0.003490658503988666988 ) ;
#1915=CARTESIAN_POINT ( 'NONE',  ( 2.949999999999943334, 2.500000000000000000, 6.495190528383297135 ) ) ;
#1916=EDGE_LOOP ( 'NONE', ( #32518, #36802 ) ) ;
#1917=ORIENTED_EDGE ( 'NONE', *, *, #91979, .T. ) ;
#1918=DIRECTION ( 'NONE',  ( -0.000000000000000000, 1.000000000000000000, -0.000000000000000000 ) ) ;
#1919=EDGE_CURVE ( 'NONE', #121644, #26032, #51747, .T. ) ;
#1920=DIRECTION ( 'NONE',  ( -0.000000000000000000, 1.000000000000000000, -0.000000000000000000 ) ) ;
#1921=FACE_BOUND ( 'NONE', #34728, .T. ) ;
#1922=CARTESIAN_POINT ( 'NONE',  ( 7.049999999999926992, 2.500000000000000000, 2.265063509461097357 ) ) ;
#1923=CIRCLE ( 'NONE', #123123, 0.09999999999999982514 ) ;
#1924=AXIS2_PLACEMENT_3D ( 'NONE', #114998, #124843, #3777 ) ;
#1925=AXIS2_PLACEMENT_3D ( 'NONE', #19700, #117881, #28232 ) ;
#1926=EDGE_LOOP ( 'NONE', ( #31248, #128784 ) ) ;
#1927=CARTESIAN_POINT ( 'NONE',  ( 6.899999999999928413, 12.50000000000000000, 4.676537180435972552 ) ) ;
#1929=AXIS2_PLACEMENT_3D ( 'NONE', #81457, #102386, #61166 ) ;
#1930=ORIENTED_EDGE ( 'NONE', *, *, #113657, .F. ) ;
#1931=CARTESIAN_POINT ( 'NONE',  ( -13.14999999999999147, 2.500000000000000000, 1.818653347947325472 ) ) ;
#1932=PLANE ( 'NONE',  #55460 ) ;
#1933=VECTOR ( 'NONE', #87660, 1000.000000000000000 ) ;
#1934=EDGE_LOOP ( 'NONE', ( #126264, #112449 ) ) ;
#1935=DIRECTION ( 'NONE',  ( 0.000000000000000000, 0.000000000000000000, 1.000000000000000000 ) ) ;
#1936=FACE_OUTER_BOUND ( 'NONE', #34415, .T. ) ;
#1937=ORIENTED_EDGE ( 'NONE', *, *, #30650, .F. ) ;
#1938=ADVANCED_FACE ( 'NONE', ( #81831 ), #7918, .T. ) ;
#1939=LINE ( 'NONE', #90311, #82223 ) ;
#1940=CARTESIAN_POINT ( 'NONE',  ( -15.39999999999997904, 12.50000000000000000, -0.06509327318403743123 ) ) ;
#1943=EDGE_LOOP ( 'NONE', ( #79197, #1963, #90048, #4280 ) ) ;
#1944=EDGE_LOOP ( 'NONE', ( #6201, #74544, #26451, #49616 ) ) ;
#1945=DIRECTION ( 'NONE',  ( 0.000000000000000000, -0.9999939076577903929, 0.003490651415223739937 ) ) ;
#1946=EDGE_CURVE ( 'NONE', #118122, #5223, #20455, .T. ) ;
#1947=ORIENTED_EDGE ( 'NONE', *, *, #126529, .F. ) ;
#1948=CARTESIAN_POINT ( 'NONE',  ( 14.59999999999989484, 2.500000000000000000, 0.6928203230275494784 ) ) ;
#1949=CARTESIAN_POINT ( 'NONE',  ( 11.24999999999990763, 2.500000000000000000, -7.288010851410854585 ) ) ;
#1950=DIRECTION ( 'NONE',  ( -0.000000000000000000, 1.000000000000000000, -0.000000000000000000 ) ) ;
#1951=EDGE_LOOP ( 'NONE', ( #35179, #119082 ) ) ;
#1953=DIRECTION ( 'NONE',  ( 0.000000000000000000, 0.000000000000000000, -1.000000000000000000 ) ) ;
#1954=CARTESIAN_POINT ( 'NONE',  ( -6.850000000000017408, 2.500000000000000000, -6.741600689897077281 ) ) ;
#1955=EDGE_CURVE ( 'NONE', #42274, #129541, #12445, .T. ) ;
#1956=EDGE_CURVE ( 'NONE', #7039, #31303, #74832, .T. ) ;
#1957=DIRECTION ( 'NONE',  ( 0.000000000000000000, 0.000000000000000000, 1.000000000000000000 ) ) ;
#1958=DIRECTION ( 'NONE',  ( 0.000000000000000000, 1.000000000000000000, 0.000000000000000000 ) ) ;
#1959=ADVANCED_FACE ( 'NONE', ( #40659 ), #110026, .T. ) ;
#1960=ADVANCED_FACE ( 'NONE', ( #80568 ), #104080, .T. ) ;
#1961=CONICAL_SURFACE ( 'NONE', #83468, 0.1000000000000002554, 0.003490658503988666988 ) ;
#1962=CARTESIAN_POINT ( 'NONE',  ( -10.80000000000000071, 2.500000000000000000, -2.276824562219559311E-15 ) ) ;
#1963=ORIENTED_EDGE ( 'NONE', *, *, #82838, .F. ) ;
#1964=VERTEX_POINT ( 'NONE', #61578 ) ;
#1965=PLANE ( 'NONE',  #20225 ) ;
#1968=EDGE_LOOP ( 'NONE', ( #32474, #90546, #56776, #69502 ) ) ;
#1969=VERTEX_POINT ( 'NONE', #22303 ) ;
#1970=ORIENTED_EDGE ( 'NONE', *, *, #23266, .T. ) ;
#1971=VECTOR ( 'NONE', #36293, 1000.000000000000000 ) ;
#1972=EDGE_CURVE ( 'NONE', #59884, #29149, #122425, .T. ) ;
#1973=FACE_OUTER_BOUND ( 'NONE', #96621, .T. ) ;
#1974=ADVANCED_FACE ( 'NONE', ( #102133 ), #95199, .T. ) ;
#1975=CARTESIAN_POINT ( 'NONE',  ( -4.350000000000023626, 12.50000000000000000, 6.841600689897072485 ) ) ;
#1976=EDGE_CURVE ( 'NONE', #29091, #11967, #22049, .T. ) ;
#1977=CARTESIAN_POINT ( 'NONE',  ( -4.550000000000022915, 2.500000000000000000, -2.065063509461102065 ) ) ;
#1979=VECTOR ( 'NONE', #7005, 1000.000000000000000 ) ;
#1980=DIRECTION ( 'NONE',  ( 0.000000000000000000, -0.000000000000000000, 1.000000000000000000 ) ) ;
#1981=FACE_OUTER_BOUND ( 'NONE', #28031, .T. ) ;
#1982=CARTESIAN_POINT ( 'NONE',  ( -4.800000000000024691, 2.500000000000000000, 0.2464101615137735679 ) ) ;
#1983=CARTESIAN_POINT ( 'NONE',  ( 8.349999999999919709, 2.500000000000000000, -2.165063509461101710 ) ) ;
#1984=LINE ( 'NONE', #3287, #46618 ) ;
#1985=AXIS2_PLACEMENT_3D ( 'NONE', #76175, #47358, #75510 ) ;
#1987=DIRECTION ( 'NONE',  ( 0.000000000000000000, 0.000000000000000000, 1.000000000000000000 ) ) ;
#1988=AXIS2_PLACEMENT_3D ( 'NONE', #48885, #88791, #39075 ) ;
#1989=CIRCLE ( 'NONE', #106542, 0.1000000000000002554 ) ;
#1990=ORIENTED_EDGE ( 'NONE', *, *, #37165, .T. ) ;
#1991=CARTESIAN_POINT ( 'NONE',  ( 9.549999999999918998, 12.50000000000000000, -6.495190528383302464 ) ) ;
#1993=VERTEX_POINT ( 'NONE', #32772 ) ;
#1994=CARTESIAN_POINT ( 'NONE',  ( -9.350000000000008527, 2.500000000000000000, -6.148780366869520897 ) ) ;
#1995=DIRECTION ( 'NONE',  ( -0.000000000000000000, 1.000000000000000000, -0.000000000000000000 ) ) ;
#1996=DIRECTION ( 'NONE',  ( -0.000000000000000000, -1.000000000000000000, -0.000000000000000000 ) ) ;
#1997=CARTESIAN_POINT ( 'NONE',  ( -12.29999999999999538, 12.50000000000000000, 4.676537180435972552 ) ) ;
#1998=DIRECTION ( 'NONE',  ( -0.000000000000000000, 1.000000000000000000, -0.000000000000000000 ) ) ;
#1999=DIRECTION ( 'NONE',  ( 0.000000000000000000, 0.000000000000000000, -1.000000000000000000 ) ) ;
#2000=DIRECTION ( 'NONE',  ( 0.000000000000000000, 0.000000000000000000, 1.000000000000000000 ) ) ;
#2001=CONICAL_SURFACE ( 'NONE', #118989, 0.1000000000000000056, 0.003490658503988666988 ) ;
#2002=ORIENTED_EDGE ( 'NONE', *, *, #98816, .T. ) ;
#2003=ORIENTED_EDGE ( 'NONE', *, *, #62084, .T. ) ;
#2004=VECTOR ( 'NONE', #262, 1000.000000000000000 ) ;
#2005=AXIS2_PLACEMENT_3D ( 'NONE', #37136, #18764, #126145 ) ;
#2006=EDGE_LOOP ( 'NONE', ( #52260, #56304 ) ) ;
#2007=ORIENTED_EDGE ( 'NONE', *, *, #55189, .T. ) ;
#2008=ADVANCED_FACE ( 'NONE', ( #72675 ), #112602, .T. ) ;
#2009=ORIENTED_EDGE ( 'NONE', *, *, #69256, .T. ) ;
#2010=LINE ( 'NONE', #81858, #10583 ) ;
#2011=AXIS2_PLACEMENT_3D ( 'NONE', #76092, #107487, #6042 ) ;
#2012=DIRECTION ( 'NONE',  ( 0.000000000000000000, 0.000000000000000000, 1.000000000000000000 ) ) ;
#2014=CONICAL_SURFACE ( 'NONE', #75188, 0.1000000000000002554, 0.003490658503988666988 ) ;
#2015=ADVANCED_FACE ( 'NONE', ( #79910 ), #17816, .T. ) ;
#2016=CARTESIAN_POINT ( 'NONE',  ( 10.59999999999990905, 12.50000000000000000, -4.676537180435978769 ) ) ;
#2017=DIRECTION ( 'NONE',  ( -0.000000000000000000, -1.000000000000000000, -0.000000000000000000 ) ) ;
#2018=EDGE_CURVE ( 'NONE', #110215, #88657, #24093, .T. ) ;
#2019=DIRECTION ( 'NONE',  ( -0.000000000000000000, -1.000000000000000000, -0.000000000000000000 ) ) ;
#2020=VERTEX_POINT ( 'NONE', #70098 ) ;
#2021=DIRECTION ( 'NONE',  ( -0.000000000000000000, 1.000000000000000000, -0.000000000000000000 ) ) ;
#2022=DIRECTION ( 'NONE',  ( 0.000000000000000000, 0.000000000000000000, 1.000000000000000000 ) ) ;
#2023=CARTESIAN_POINT ( 'NONE',  ( 4.149999999999939959, 2.500000000000000000, 1.472243186433545459 ) ) ;
#2024=LINE ( 'NONE', #30873, #24273 ) ;
#2025=AXIS2_PLACEMENT_3D ( 'NONE', #23024, #54404, #123157 ) ;
#2026=EDGE_CURVE ( 'NONE', #29271, #62565, #20350, .T. ) ;
#2027=CARTESIAN_POINT ( 'NONE',  ( -0.6000000000000383915, 2.500000000000000000, -3.983716857408426293 ) ) ;
#2028=AXIS2_PLACEMENT_3D ( 'NONE', #8140, #64017, #45034 ) ;
#2029=ORIENTED_EDGE ( 'NONE', *, *, #71569, .T. ) ;
#2030=VECTOR ( 'NONE', #116044, 1000.000000000000000 ) ;
#2031=EDGE_LOOP ( 'NONE', ( #104443, #44555 ) ) ;
#2032=ORIENTED_EDGE ( 'NONE', *, *, #21171, .T. ) ;
#2033=DIRECTION ( 'NONE',  ( 0.000000000000000000, 0.000000000000000000, 1.000000000000000000 ) ) ;
#2034=ORIENTED_EDGE ( 'NONE', *, *, #3891, .T. ) ;
#2035=CIRCLE ( 'NONE', #108649, 0.1000000000000000056 ) ;
#2036=DIRECTION ( 'NONE',  ( 0.000000000000000000, 1.000000000000000000, 0.000000000000000000 ) ) ;
#2037=CARTESIAN_POINT ( 'NONE',  ( 2.949999999999946887, 12.50000000000000000, -6.495190528383302464 ) ) ;
#2038=CIRCLE ( 'NONE', #62708, 0.09999999999999982514 ) ;
#2039=EDGE_LOOP ( 'NONE', ( #78932, #71187, #48499, #34133 ) ) ;
#2040=CARTESIAN_POINT ( 'NONE',  ( -3.749999999999991118, 2.500000000000000000, -2.165063509461101710 ) ) ;
#2041=DIRECTION ( 'NONE',  ( 0.000000000000000000, 0.000000000000000000, 1.000000000000000000 ) ) ;
#2042=DIRECTION ( 'NONE',  ( 0.000000000000000000, 0.000000000000000000, 1.000000000000000000 ) ) ;
#2043=EDGE_CURVE ( 'NONE', #116823, #102121, #53346, .T. ) ;
#2044=DIRECTION ( 'NONE',  ( 0.000000000000000000, 1.000000000000000000, 0.000000000000000000 ) ) ;
#2045=DIRECTION ( 'NONE',  ( 0.000000000000000000, -0.000000000000000000, 1.000000000000000000 ) ) ;
#2047=ORIENTED_EDGE ( 'NONE', *, *, #103340, .F. ) ;
#2048=DIRECTION ( 'NONE',  ( 0.000000000000000000, 0.000000000000000000, 1.000000000000000000 ) ) ;
#2049=DIRECTION ( 'NONE',  ( 0.000000000000000000, 1.000000000000000000, 0.000000000000000000 ) ) ;
#2050=DIRECTION ( 'NONE',  ( 0.000000000000000000, 1.000000000000000000, 0.000000000000000000 ) ) ;
#2051=CARTESIAN_POINT ( 'NONE',  ( 6.649999999999929301, 12.50000000000000000, -2.230156782645139391 ) ) ;
#2052=ORIENTED_EDGE ( 'NONE', *, *, #17167, .F. ) ;
#2053=EDGE_CURVE ( 'NONE', #16443, #71159, #109772, .T. ) ;
#2054=ORIENTED_EDGE ( 'NONE', *, *, #108201, .T. ) ;
#2055=DIRECTION ( 'NONE',  ( 0.000000000000000000, 0.000000000000000000, 1.000000000000000000 ) ) ;
#2056=AXIS2_PLACEMENT_3D ( 'NONE', #75866, #74588, #114501 ) ;
#2057=CARTESIAN_POINT ( 'NONE',  ( -3.150000000000029221, 2.500000000000000000, -1.718653347947326049 ) ) ;
#2058=DIRECTION ( 'NONE',  ( 0.000000000000000000, 0.000000000000000000, 1.000000000000000000 ) ) ;
#2059=DIRECTION ( 'NONE',  ( 0.000000000000000000, -0.9999939076577903929, 0.003490651415223739937 ) ) ;
#2060=EDGE_LOOP ( 'NONE', ( #72816, #22527, #87175, #90661 ) ) ;
#2061=DIRECTION ( 'NONE',  ( -0.000000000000000000, 1.000000000000000000, -0.000000000000000000 ) ) ;
#2062=VECTOR ( 'NONE', #123414, 1000.000000000000000 ) ;
#2063=AXIS2_PLACEMENT_3D ( 'NONE', #22709, #23318, #114286 ) ;
#2064=DIRECTION ( 'NONE',  ( 0.000000000000000000, 0.000000000000000000, 1.000000000000000000 ) ) ;
#2065=ORIENTED_EDGE ( 'NONE', *, *, #105794, .F. ) ;
#2066=DIRECTION ( 'NONE',  ( 0.000000000000000000, 0.000000000000000000, 1.000000000000000000 ) ) ;
#2067=EDGE_CURVE ( 'NONE', #69989, #11966, #9427, .T. ) ;
#2068=EDGE_LOOP ( 'NONE', ( #577, #22664 ) ) ;
#2070=AXIS2_PLACEMENT_3D ( 'NONE', #54502, #104260, #34251 ) ;
#2071=CIRCLE ( 'NONE', #5991, 0.06509327318403745899 ) ;
#2073=DIRECTION ( 'NONE',  ( -0.000000000000000000, 1.000000000000000000, -0.000000000000000000 ) ) ;
#2075=ORIENTED_EDGE ( 'NONE', *, *, #123890, .T. ) ;
#2076=EDGE_CURVE ( 'NONE', #126002, #109254, #61763, .T. ) ;
#2077=ORIENTED_EDGE ( 'NONE', *, *, #65642, .T. ) ;
#2078=LINE ( 'NONE', #10597, #125064 ) ;
#2079=DIRECTION ( 'NONE',  ( -0.000000000000000000, 1.000000000000000000, -0.000000000000000000 ) ) ;
#2083=DIRECTION ( 'NONE',  ( -4.274815082592931898E-19, -0.9999939076577903929, -0.003490651415223739937 ) ) ;
#2084=DIRECTION ( 'NONE',  ( -0.000000000000000000, 1.000000000000000000, -0.000000000000000000 ) ) ;
#2085=CARTESIAN_POINT ( 'NONE',  ( -4.200000000000025935, 2.500000000000000000, 4.430127018922196847 ) ) ;
#2086=DIRECTION ( 'NONE',  ( -0.000000000000000000, 1.000000000000000000, -0.000000000000000000 ) ) ;
#2087=CIRCLE ( 'NONE', #98244, 0.1000000000000002554 ) ;
#2088=CIRCLE ( 'NONE', #46039, 0.06509327318403745899 ) ;
#2089=VERTEX_POINT ( 'NONE', #45796 ) ;
#2090=EDGE_CURVE ( 'NONE', #56145, #82216, #19899, .T. ) ;
#2091=ORIENTED_EDGE ( 'NONE', *, *, #119329, .T. ) ;
#2092=DIRECTION ( 'NONE',  ( 0.000000000000000000, 0.000000000000000000, 1.000000000000000000 ) ) ;
#2093=EDGE_LOOP ( 'NONE', ( #26547, #67364 ) ) ;
#2094=LINE ( 'NONE', #11278, #78879 ) ;
#2095=DIRECTION ( 'NONE',  ( -0.000000000000000000, 1.000000000000000000, -0.000000000000000000 ) ) ;
#2096=CARTESIAN_POINT ( 'NONE',  ( 11.24999999999990941, 2.500000000000000000, 7.288010851410849256 ) ) ;
#2097=ORIENTED_EDGE ( 'NONE', *, *, #86362, .T. ) ;
#2098=VERTEX_POINT ( 'NONE', #55605 ) ;
#2099=FACE_BOUND ( 'NONE', #82400, .T. ) ;
#2100=EDGE_LOOP ( 'NONE', ( #12731, #84755, #61103, #86237 ) ) ;
#2101=CARTESIAN_POINT ( 'NONE',  ( -7.050000000000016698, 2.500000000000000000, -6.495190528383302464 ) ) ;
#2102=DIRECTION ( 'NONE',  ( 0.000000000000000000, 0.000000000000000000, -1.000000000000000000 ) ) ;
#2103=AXIS2_PLACEMENT_3D ( 'NONE', #1888, #117953, #109928 ) ;
#2104=LINE ( 'NONE', #93725, #17844 ) ;
#2105=ADVANCED_FACE ( 'NONE', ( #13732 ), #114512, .T. ) ;
#2106=DIRECTION ( 'NONE',  ( 0.000000000000000000, -0.9999939076577903929, 0.003490651415223739937 ) ) ;
#2107=CARTESIAN_POINT ( 'NONE',  ( -14.34999999999998543, 2.500000000000000000, -1.818653347947323695 ) ) ;
#2108=FACE_OUTER_BOUND ( 'NONE', #7305, .T. ) ;
#2109=PLANE ( 'NONE',  #51899 ) ;
#2110=CARTESIAN_POINT ( 'NONE',  ( -6.050000000000022027, 12.50000000000000000, -1.818653347947326138 ) ) ;
#2111=EDGE_CURVE ( 'NONE', #114814, #54801, #54954, .T. ) ;
#2112=ADVANCED_FACE ( 'NONE', ( #94884 ), #42900, .T. ) ;
#2113=DIRECTION ( 'NONE',  ( 0.000000000000000000, 0.000000000000000000, 1.000000000000000000 ) ) ;
#2114=CARTESIAN_POINT ( 'NONE',  ( 0.3999999999999568345, 12.50000000000000000, -5.088040615133791356 ) ) ;
#2115=ADVANCED_FACE ( 'NONE', ( #5198 ), #13609, .T. ) ;
#2116=AXIS2_PLACEMENT_3D ( 'NONE', #32554, #1129, #12858 ) ;
#2117=EDGE_CURVE ( 'NONE', #59989, #16485, #36632, .T. ) ;
#2118=DIRECTION ( 'NONE',  ( -0.000000000000000000, -1.000000000000000000, -0.000000000000000000 ) ) ;
#2119=AXIS2_PLACEMENT_3D ( 'NONE', #116659, #105564, #7342 ) ;
#2120=ORIENTED_EDGE ( 'NONE', *, *, #123129, .F. ) ;
#2121=EDGE_LOOP ( 'NONE', ( #99318, #70918, #55112, #35769 ) ) ;
#2122=AXIS2_PLACEMENT_3D ( 'NONE', #49903, #9959, #102214 ) ;
#2123=ORIENTED_EDGE ( 'NONE', *, *, #1805, .F. ) ;
#2124=DIRECTION ( 'NONE',  ( 0.000000000000000000, 0.000000000000000000, -1.000000000000000000 ) ) ;
#2125=VERTEX_POINT ( 'NONE', #45157 ) ;
#2126=DIRECTION ( 'NONE',  ( -0.000000000000000000, 1.000000000000000000, -0.000000000000000000 ) ) ;
#2127=EDGE_CURVE ( 'NONE', #6598, #3681, #116024, .T. ) ;
#2128=FACE_OUTER_BOUND ( 'NONE', #86643, .T. ) ;
#2129=EDGE_CURVE ( 'NONE', #10801, #33059, #70061, .T. ) ;
#2131=ORIENTED_EDGE ( 'NONE', *, *, #4841, .T. ) ;
#2132=EDGE_LOOP ( 'NONE', ( #51989, #93357, #36210, #32245 ) ) ;
#2133=ADVANCED_FACE ( 'NONE', ( #75240 ), #59622, .T. ) ;
#2134=CARTESIAN_POINT ( 'NONE',  ( -9.400000000000007461, 12.50000000000000000, 4.611443907251934426 ) ) ;
#2135=AXIS2_PLACEMENT_3D ( 'NONE', #18953, #80492, #79199 ) ;
#2136=EDGE_CURVE ( 'NONE', #77027, #10762, #44491, .T. ) ;
#2137=ADVANCED_FACE ( 'NONE', ( #73958 ), #57546, .T. ) ;
#2138=CARTESIAN_POINT ( 'NONE',  ( -0.4000000000000401013, 2.500000000000000000, -3.537306695894649966 ) ) ;
#2139=CARTESIAN_POINT ( 'NONE',  ( -3.750000000000031086, 12.50000000000000000, -5.802370205355749988 ) ) ;
#2140=CARTESIAN_POINT ( 'NONE',  ( -10.00000000000000711, 2.500000000000000000, -3.737306695894645259 ) ) ;
#2141=CIRCLE ( 'NONE', #29349, 0.1000000000000002554 ) ;
#2142=CARTESIAN_POINT ( 'NONE',  ( -7.050000000000016698, 2.500000000000000000, -2.265063509461101798 ) ) ;
#2143=CARTESIAN_POINT ( 'NONE',  ( 3.749999999999942268, 2.500000000000000000, -5.902370205355750521 ) ) ;
#2144=EDGE_LOOP ( 'NONE', ( #12589, #99223 ) ) ;
#2145=EDGE_CURVE ( 'NONE', #112302, #40817, #26153, .T. ) ;
#2146=DIRECTION ( 'NONE',  ( 0.000000000000000000, -0.9999939076577903929, 0.003490651415223739937 ) ) ;
#2147=VERTEX_POINT ( 'NONE', #4536 ) ;
#2149=ORIENTED_EDGE ( 'NONE', *, *, #71143, .T. ) ;
#2150=DIRECTION ( 'NONE',  ( 0.000000000000000000, 0.000000000000000000, -1.000000000000000000 ) ) ;
#2151=ORIENTED_EDGE ( 'NONE', *, *, #94338, .T. ) ;
#2152=ORIENTED_EDGE ( 'NONE', *, *, #11842, .F. ) ;
#2153=ORIENTED_EDGE ( 'NONE', *, *, #30560, .F. ) ;
#2154=LINE ( 'NONE', #100369, #90385 ) ;
#2155=CARTESIAN_POINT ( 'NONE',  ( -11.84999999999999787, 2.500000000000000000, -2.511473670974873951 ) ) ;
#2156=DIRECTION ( 'NONE',  ( 0.000000000000000000, 0.000000000000000000, -1.000000000000000000 ) ) ;
#2157=FACE_OUTER_BOUND ( 'NONE', #5443, .T. ) ;
#2158=LINE ( 'NONE', #61090, #65860 ) ;
#2159=CIRCLE ( 'NONE', #96232, 0.06509327318403745899 ) ;
#2161=CONICAL_SURFACE ( 'NONE', #4204, 0.1000000000000002554, 0.003490658503988666988 ) ;
#2162=DIRECTION ( 'NONE',  ( 0.000000000000000000, 0.000000000000000000, -1.000000000000000000 ) ) ;
#2163=ORIENTED_EDGE ( 'NONE', *, *, #93567, .T. ) ;
#2164=CARTESIAN_POINT ( 'NONE',  ( 9.149999999999918643, 12.50000000000000000, -6.495190528383302464 ) ) ;
#2165=AXIS2_PLACEMENT_3D ( 'NONE', #45371, #33609, #25070 ) ;
#2166=CIRCLE ( 'NONE', #35633, 0.1000000000000002554 ) ;
#2167=ORIENTED_EDGE ( 'NONE', *, *, #97078, .T. ) ;
#2168=CARTESIAN_POINT ( 'NONE',  ( 1.649999999999951950, 2.500000000000000000, -5.702370205355749455 ) ) ;
#2169=ORIENTED_EDGE ( 'NONE', *, *, #19435, .F. ) ;
#2170=DIRECTION ( 'NONE',  ( -0.000000000000000000, 1.000000000000000000, -0.000000000000000000 ) ) ;
#2173=EDGE_CURVE ( 'NONE', #76, #94866, #40844, .T. ) ;
#2174=CARTESIAN_POINT ( 'NONE',  ( 10.44999999999991047, 12.50000000000000000, -6.430097255199264339 ) ) ;
#2175=ADVANCED_FACE ( 'NONE', ( #73301 ), #111918, .T. ) ;
#2176=EDGE_LOOP ( 'NONE', ( #95967, #28992 ) ) ;
#2177=EDGE_LOOP ( 'NONE', ( #104373, #50226 ) ) ;
#2178=CARTESIAN_POINT ( 'NONE',  ( -7.900000000000014566, 2.500000000000000000, -4.922947341949753586 ) ) ;
#2179=FACE_OUTER_BOUND ( 'NONE', #77936, .T. ) ;
#2180=CARTESIAN_POINT ( 'NONE',  ( -5.200000000000020606, 12.50000000000000000, 3.983716857408420964 ) ) ;
#2181=DIRECTION ( 'NONE',  ( 0.000000000000000000, 0.000000000000000000, 1.000000000000000000 ) ) ;
#2182=EDGE_CURVE ( 'NONE', #9827, #97225, #122304, .T. ) ;
#2183=DIRECTION ( 'NONE',  ( 0.000000000000000000, 1.000000000000000000, 0.000000000000000000 ) ) ;
#2184=EDGE_LOOP ( 'NONE', ( #6771, #10215 ) ) ;
#2185=CARTESIAN_POINT ( 'NONE',  ( -14.59999999999998366, 12.50000000000000000, 0.6928203230275518099 ) ) ;
#2186=ORIENTED_EDGE ( 'NONE', *, *, #13563, .F. ) ;
#2187=DIRECTION ( 'NONE',  ( 0.000000000000000000, 1.000000000000000000, 0.000000000000000000 ) ) ;
#2188=CARTESIAN_POINT ( 'NONE',  ( 14.79999999999989235, 2.500000000000000000, 0.3464101615137735735 ) ) ;
#2189=VECTOR ( 'NONE', #5687, 1000.000000000000000 ) ;
#2190=FACE_OUTER_BOUND ( 'NONE', #87131, .T. ) ;
#2191=FACE_OUTER_BOUND ( 'NONE', #19020, .T. ) ;
#2192=DIRECTION ( 'NONE',  ( 0.000000000000000000, 1.000000000000000000, 0.000000000000000000 ) ) ;
#2194=DIRECTION ( 'NONE',  ( 0.000000000000000000, 1.000000000000000000, 0.000000000000000000 ) ) ;
#2195=VERTEX_POINT ( 'NONE', #66702 ) ;
#2196=CIRCLE ( 'NONE', #90019, 0.06509327318403745899 ) ;
#2197=DIRECTION ( 'NONE',  ( -0.000000000000000000, -1.000000000000000000, -0.000000000000000000 ) ) ;
#2198=DIRECTION ( 'NONE',  ( 0.000000000000000000, 1.000000000000000000, 0.000000000000000000 ) ) ;
#2199=DIRECTION ( 'NONE',  ( 0.000000000000000000, -0.000000000000000000, 1.000000000000000000 ) ) ;
#2200=ORIENTED_EDGE ( 'NONE', *, *, #44168, .T. ) ;
#2201=EDGE_LOOP ( 'NONE', ( #109300, #34604 ) ) ;
#2202=DIRECTION ( 'NONE',  ( 0.000000000000000000, 1.000000000000000000, 0.000000000000000000 ) ) ;
#2203=EDGE_CURVE ( 'NONE', #91908, #127901, #38787, .T. ) ;
#2204=VECTOR ( 'NONE', #106545, 1000.000000000000000 ) ;
#2205=ORIENTED_EDGE ( 'NONE', *, *, #63753, .T. ) ;
#2206=B_SPLINE_SURFACE_WITH_KNOTS ( 'NONE', 3, 1, ( 
 ( #98243, #108068 ),
 ( #128385, #119182 ),
 ( #44, #90347 ),
 ( #59652, #10501 ),
 ( #70725, #79900 ),
 ( #70088, #58979 ),
 ( #110016, #110646 ),
 ( #58348, #98889 ),
 ( #20342, #30826 ),
 ( #60291, #20978 ) ),
 .UNSPECIFIED., .F., .F., .F.,
 ( 4, 2, 2, 2, 4 ),
 ( 2, 2 ),
 ( 0.000000000000000000, 0.2500000000000000555, 0.5000000000000001110, 0.7500000000000000000, 1.000000000000000000 ),
 ( 0.000000000000000000, 1.000000000000000000 ),
 .UNSPECIFIED. ) ;
#2207=VERTEX_POINT ( 'NONE', #28734 ) ;
#2208=FACE_OUTER_BOUND ( 'NONE', #5583, .T. ) ;
#2209=ORIENTED_EDGE ( 'NONE', *, *, #56633, .T. ) ;
#2210=CARTESIAN_POINT ( 'NONE',  ( 18.98912670146303938, -2.543039972612231026, -4.488908218021264496 ) ) ;
#2211=DIRECTION ( 'NONE',  ( 0.000000000000000000, 1.000000000000000000, 0.000000000000000000 ) ) ;
#2212=CARTESIAN_POINT ( 'NONE',  ( 20.37025966759629725, 0.6621301594407191793, 4.188616773932410275 ) ) ;
#2213=CONICAL_SURFACE ( 'NONE', #14809, 0.1000000000000002554, 0.003490658503988666988 ) ;
#2214=ORIENTED_EDGE ( 'NONE', *, *, #2357, .T. ) ;
#2215=DIRECTION ( 'NONE',  ( 0.000000000000000000, 1.000000000000000000, 0.000000000000000000 ) ) ;
#2216=DIRECTION ( 'NONE',  ( 0.000000000000000000, 0.000000000000000000, -1.000000000000000000 ) ) ;
#2217=CIRCLE ( 'NONE', #56591, 0.06509327318403745899 ) ;
#2218=ADVANCED_FACE ( 'NONE', ( #67322 ), #55487, .T. ) ;
#2219=EDGE_CURVE ( 'NONE', #58977, #67840, #113971, .T. ) ;
#2220=VERTEX_POINT ( 'NONE', #58830 ) ;
#2221=EDGE_LOOP ( 'NONE', ( #51847, #87279, #93317, #109129 ) ) ;
#2222=ORIENTED_EDGE ( 'NONE', *, *, #29947, .T. ) ;
#2223=DIRECTION ( 'NONE',  ( -0.000000000000000000, -1.000000000000000000, -0.000000000000000000 ) ) ;
#2224=DIRECTION ( 'NONE',  ( 0.000000000000000000, 1.000000000000000000, 0.000000000000000000 ) ) ;
#2225=CARTESIAN_POINT ( 'NONE',  ( 5.649999999999934630, 12.50000000000000000, -1.818653347947325916 ) ) ;
#2226=EDGE_CURVE ( 'NONE', #87462, #63696, #69273, .T. ) ;
#2227=FACE_BOUND ( 'NONE', #42197, .T. ) ;
#2228=EDGE_LOOP ( 'NONE', ( #117663, #107045, #105670, #22259 ) ) ;
#2229=DIRECTION ( 'NONE',  ( -0.000000000000000000, 1.000000000000000000, -0.000000000000000000 ) ) ;
#2230=CARTESIAN_POINT ( 'NONE',  ( 6.249999999999928946, 12.50000000000000000, 2.792790559304612064 ) ) ;
#2231=ORIENTED_EDGE ( 'NONE', *, *, #19266, .T. ) ;
#2232=DIRECTION ( 'NONE',  ( -4.274815082592931898E-19, -0.9999939076577903929, -0.003490651415223739937 ) ) ;
#2233=DIRECTION ( 'NONE',  ( 0.000000000000000000, 0.000000000000000000, -1.000000000000000000 ) ) ;
#2234=VECTOR ( 'NONE', #76226, 1000.000000000000000 ) ;
#2235=DIRECTION ( 'NONE',  ( 0.000000000000000000, 1.000000000000000000, 0.000000000000000000 ) ) ;
#2236=CARTESIAN_POINT ( 'NONE',  ( 3.749999999999942268, 2.500000000000000000, -5.802370205355749988 ) ) ;
#2237=CARTESIAN_POINT ( 'NONE',  ( 6.049999999999932321, 2.500000000000000000, 1.718653347947321386 ) ) ;
#2238=CIRCLE ( 'NONE', #185, 0.1000000000000002554 ) ;
#2239=AXIS2_PLACEMENT_3D ( 'NONE', #129365, #18081, #57375 ) ;
#2240=DIRECTION ( 'NONE',  ( -0.000000000000000000, -1.000000000000000000, -0.000000000000000000 ) ) ;
#2241=DIRECTION ( 'NONE',  ( 0.000000000000000000, 0.000000000000000000, -1.000000000000000000 ) ) ;
#2242=AXIS2_PLACEMENT_3D ( 'NONE', #15885, #95748, #76106 ) ;
#2243=EDGE_LOOP ( 'NONE', ( #9958, #124399, #108955, #90283 ) ) ;
#2244=EDGE_LOOP ( 'NONE', ( #111426, #90679, #74627, #129328 ) ) ;
#2245=EDGE_LOOP ( 'NONE', ( #34887, #68094, #50064, #123822 ) ) ;
#2246=ORIENTED_EDGE ( 'NONE', *, *, #28925, .T. ) ;
#2247=DIRECTION ( 'NONE',  ( -4.274815082592931898E-19, -0.9999939076577903929, -0.003490651415223739937 ) ) ;
#2248=CARTESIAN_POINT ( 'NONE',  ( -10.40000000000000213, 2.500000000000000000, -5.122947341949750211 ) ) ;
#2249=AXIS2_PLACEMENT_3D ( 'NONE', #82818, #122094, #32446 ) ;
#2250=LINE ( 'NONE', #112229, #61372 ) ;
#2251=VERTEX_POINT ( 'NONE', #36630 ) ;
#2252=FACE_BOUND ( 'NONE', #106027, .T. ) ;
#2253=CARTESIAN_POINT ( 'NONE',  ( -13.74999999999995381, 12.50000000000000000, -2.165063509461099489 ) ) ;
#2254=CARTESIAN_POINT ( 'NONE',  ( -13.34999999999999076, 12.50000000000000000, -2.165063509461099489 ) ) ;
#2255=CARTESIAN_POINT ( 'NONE',  ( 4.349999999999941025, 12.50000000000000000, -1.818653347947326138 ) ) ;
#2256=EDGE_CURVE ( 'NONE', #70431, #9486, #15752, .T. ) ;
#2257=CARTESIAN_POINT ( 'NONE',  ( 0.5999999999999555689, 2.500000000000000000, 4.676537180435972552 ) ) ;
#2258=FACE_OUTER_BOUND ( 'NONE', #54075, .T. ) ;
#2259=DIRECTION ( 'NONE',  ( 0.000000000000000000, 1.000000000000000000, 0.000000000000000000 ) ) ;
#2260=FACE_OUTER_BOUND ( 'NONE', #8307, .T. ) ;
#2261=DIRECTION ( 'NONE',  ( -0.000000000000000000, -1.000000000000000000, -0.000000000000000000 ) ) ;
#2263=DIRECTION ( 'NONE',  ( 0.000000000000000000, 1.000000000000000000, 0.000000000000000000 ) ) ;
#2264=EDGE_CURVE ( 'NONE', #38409, #7115, #76326, .T. ) ;
#2266=EDGE_LOOP ( 'NONE', ( #92439, #23875, #12611, #22147 ) ) ;
#2268=ORIENTED_EDGE ( 'NONE', *, *, #26548, .F. ) ;
#2269=VERTEX_POINT ( 'NONE', #58202 ) ;
#2270=EDGE_CURVE ( 'NONE', #56716, #12489, #56869, .T. ) ;
#2271=EDGE_LOOP ( 'NONE', ( #24593, #18778, #12277, #12430 ) ) ;
#2272=DIRECTION ( 'NONE',  ( 0.000000000000000000, -0.9999939076577903929, 0.003490651415223739937 ) ) ;
#2273=ADVANCED_FACE ( 'NONE', ( #56239 ), #99413, .T. ) ;
#2274=EDGE_CURVE ( 'NONE', #123488, #121393, #30466, .T. ) ;
#2275=ORIENTED_EDGE ( 'NONE', *, *, #124504, .T. ) ;
#2276=VERTEX_POINT ( 'NONE', #96804 ) ;
#2277=CIRCLE ( 'NONE', #92168, 0.06509327318403745899 ) ;
#2278=CONICAL_SURFACE ( 'NONE', #48261, 0.1000000000000000056, 0.003490658503988666988 ) ;
#2279=DIRECTION ( 'NONE',  ( -0.000000000000000000, -1.000000000000000000, -0.000000000000000000 ) ) ;
#2280=ADVANCED_FACE ( 'NONE', ( #117083 ), #86865, .T. ) ;
#2281=CARTESIAN_POINT ( 'NONE',  ( 14.18215599412843098, -2.499999999999999556, 6.639800459772741803 ) ) ;
#2282=DIRECTION ( 'NONE',  ( 0.000000000000000000, -0.9999939076577903929, 0.003490651415223739937 ) ) ;
#2283=LINE ( 'NONE', #50130, #27987 ) ;
#2284=ORIENTED_EDGE ( 'NONE', *, *, #97865, .T. ) ;
#2285=CARTESIAN_POINT ( 'NONE',  ( -9.150000000000005684, 12.50000000000000000, 5.802370205355744659 ) ) ;
#2286=EDGE_CURVE ( 'NONE', #127872, #14057, #47173, .T. ) ;
#2287=CIRCLE ( 'NONE', #110947, 0.06509327318403745899 ) ;
#2288=ORIENTED_EDGE ( 'NONE', *, *, #86039, .F. ) ;
#2289=VERTEX_POINT ( 'NONE', #38570 ) ;
#2290=CARTESIAN_POINT ( 'NONE',  ( -17.50000000000000000, 2.500000000000000000, -9.999999999999998224 ) ) ;
#2291=DIRECTION ( 'NONE',  ( 0.000000000000000000, -0.9999939076577903929, 0.003490651415223739937 ) ) ;
#2292=ORIENTED_EDGE ( 'NONE', *, *, #98914, .T. ) ;
#2293=ORIENTED_EDGE ( 'NONE', *, *, #65057, .T. ) ;
#2294=CIRCLE ( 'NONE', #92185, 0.06509327318403745899 ) ;
#2295=DIRECTION ( 'NONE',  ( 0.000000000000000000, -0.000000000000000000, 1.000000000000000000 ) ) ;
#2296=AXIS2_PLACEMENT_3D ( 'NONE', #31865, #42327, #122183 ) ;
#2297=FACE_OUTER_BOUND ( 'NONE', #63665, .T. ) ;
#2298=LINE ( 'NONE', #44833, #68775 ) ;
#2299=DIRECTION ( 'NONE',  ( -0.000000000000000000, 1.000000000000000000, -0.000000000000000000 ) ) ;
#2300=CARTESIAN_POINT ( 'NONE',  ( 12.29999999999990479, 12.50000000000000000, 4.676537180435972552 ) ) ;
#2301=CONICAL_SURFACE ( 'NONE', #88061, 0.09999999999999982514, 0.003490658503988666988 ) ;
#2302=ORIENTED_EDGE ( 'NONE', *, *, #121294, .F. ) ;
#2303=CARTESIAN_POINT ( 'NONE',  ( 7.180215335565367063, -2.500000000000000000, 8.697219394475791177 ) ) ;
#2304=ORIENTED_EDGE ( 'NONE', *, *, #62845, .F. ) ;
#2306=CARTESIAN_POINT ( 'NONE',  ( 10.39999999999990976, 2.500000000000000000, 4.330127018922196314 ) ) ;
#2307=VECTOR ( 'NONE', #80832, 1000.000000000000000 ) ;
#2308=CARTESIAN_POINT ( 'NONE',  ( 6.849999999999929479, 2.500000000000000000, 6.941600689897073018 ) ) ;
#2309=CARTESIAN_POINT ( 'NONE',  ( 4.399999999999937295, 12.50000000000000000, 4.611443907251934426 ) ) ;
#2310=FACE_OUTER_BOUND ( 'NONE', #115573, .T. ) ;
#2311=ORIENTED_EDGE ( 'NONE', *, *, #57397, .T. ) ;
#2312=DIRECTION ( 'NONE',  ( 0.000000000000000000, 0.000000000000000000, 1.000000000000000000 ) ) ;
#2313=EDGE_CURVE ( 'NONE', #28179, #11893, #24183, .T. ) ;
#2314=FACE_OUTER_BOUND ( 'NONE', #7225, .T. ) ;
#2315=EDGE_LOOP ( 'NONE', ( #116559, #35390, #114477, #73866 ) ) ;
#2316=ORIENTED_EDGE ( 'NONE', *, *, #92232, .F. ) ;
#2317=EDGE_LOOP ( 'NONE', ( #127543, #42310 ) ) ;
#2318=DIRECTION ( 'NONE',  ( 0.000000000000000000, 0.000000000000000000, 1.000000000000000000 ) ) ;
#2319=FACE_OUTER_BOUND ( 'NONE', #56475, .T. ) ;
#2321=DIRECTION ( 'NONE',  ( 0.000000000000000000, 0.000000000000000000, 1.000000000000000000 ) ) ;
#2322=CARTESIAN_POINT ( 'NONE',  ( 8.549999999999920774, 2.500000000000000000, -2.411473670974877859 ) ) ;
#2323=EDGE_CURVE ( 'NONE', #8397, #120782, #53438, .T. ) ;
#2324=FACE_OUTER_BOUND ( 'NONE', #38482, .T. ) ;
#2325=CARTESIAN_POINT ( 'NONE',  ( 7.499999999999927169, 12.50000000000000000, -5.022947341949754119 ) ) ;
#2326=DIRECTION ( 'NONE',  ( 0.000000000000000000, 0.000000000000000000, 1.000000000000000000 ) ) ;
#2327=AXIS2_PLACEMENT_3D ( 'NONE', #125629, #85073, #126943 ) ;
#2328=CIRCLE ( 'NONE', #65015, 0.1000000000000002554 ) ;
#2329=AXIS2_PLACEMENT_3D ( 'NONE', #114833, #65740, #6166 ) ;
#2330=CONICAL_SURFACE ( 'NONE', #31611, 0.09999999999999982514, 0.003490658503988666988 ) ;
#2332=ORIENTED_EDGE ( 'NONE', *, *, #69303, .F. ) ;
#2333=CARTESIAN_POINT ( 'NONE',  ( -13.09999999999999254, 12.50000000000000000, -0.3464101615137741286 ) ) ;
#2334=CONICAL_SURFACE ( 'NONE', #77658, 0.09999999999999982514, 0.003490658503988666988 ) ;
#2335=CARTESIAN_POINT ( 'NONE',  ( 4.149999999999941735, 2.500000000000000000, -2.857883832488653741 ) ) ;
#2336=DIRECTION ( 'NONE',  ( 0.000000000000000000, 0.000000000000000000, 1.000000000000000000 ) ) ;
#2337=CARTESIAN_POINT ( 'NONE',  ( 12.29999999999990656, 12.50000000000000000, -4.741630453620015118 ) ) ;
#2338=ORIENTED_EDGE ( 'NONE', *, *, #57239, .F. ) ;
#2339=FACE_OUTER_BOUND ( 'NONE', #19616, .T. ) ;
#2340=FACE_OUTER_BOUND ( 'NONE', #3049, .T. ) ;
#2341=DIRECTION ( 'NONE',  ( 0.000000000000000000, 0.000000000000000000, 1.000000000000000000 ) ) ;
#2342=ORIENTED_EDGE ( 'NONE', *, *, #12243, .F. ) ;
#2343=ORIENTED_EDGE ( 'NONE', *, *, #8656, .F. ) ;
#2344=CARTESIAN_POINT ( 'NONE',  ( 3.549999999999944755, 2.500000000000000000, -6.941600689897077459 ) ) ;
#2345=EDGE_CURVE ( 'NONE', #25156, #460, #122391, .T. ) ;
#2346=VERTEX_POINT ( 'NONE', #29383 ) ;
#2348=FACE_OUTER_BOUND ( 'NONE', #121730, .T. ) ;
#2349=CARTESIAN_POINT ( 'NONE',  ( 19.21290572970694299, 2.587129408759306859, -2.394140119531837918 ) ) ;
#2350=DIRECTION ( 'NONE',  ( -0.000000000000000000, 1.000000000000000000, -0.000000000000000000 ) ) ;
#2351=DIRECTION ( 'NONE',  ( 0.000000000000000000, 0.000000000000000000, 1.000000000000000000 ) ) ;
#2352=EDGE_CURVE ( 'NONE', #84054, #128741, #77807, .T. ) ;
#2353=ORIENTED_EDGE ( 'NONE', *, *, #36045, .F. ) ;
#2354=AXIS2_PLACEMENT_3D ( 'NONE', #77507, #126623, #67679 ) ;
#2355=DIRECTION ( 'NONE',  ( 0.000000000000000000, 1.000000000000000000, 0.000000000000000000 ) ) ;
#2356=VERTEX_POINT ( 'NONE', #20194 ) ;
#2357=EDGE_CURVE ( 'NONE', #75351, #128756, #82692, .T. ) ;
#2358=CARTESIAN_POINT ( 'NONE',  ( 6.449999999999928235, 2.500000000000000000, 2.511473670974873507 ) ) ;
#2359=DIRECTION ( 'NONE',  ( 0.000000000000000000, -0.9999939076577903929, 0.003490651415223739937 ) ) ;
#2360=EDGE_CURVE ( 'NONE', #83282, #12520, #91509, .T. ) ;
#2361=AXIS2_PLACEMENT_3D ( 'NONE', #77236, #65473, #15055 ) ;
#2362=ORIENTED_EDGE ( 'NONE', *, *, #22963, .F. ) ;
#2363=AXIS2_PLACEMENT_3D ( 'NONE', #68660, #8435, #38583 ) ;
#2364=ORIENTED_EDGE ( 'NONE', *, *, #79466, .F. ) ;
#2365=EDGE_CURVE ( 'NONE', #47194, #52167, #93148, .T. ) ;
#2366=ORIENTED_EDGE ( 'NONE', *, *, #39428, .F. ) ;
#2367=EDGE_LOOP ( 'NONE', ( #119048, #26114 ) ) ;
#2368=DIRECTION ( 'NONE',  ( 0.000000000000000000, 1.000000000000000000, 0.000000000000000000 ) ) ;
#2369=CARTESIAN_POINT ( 'NONE',  ( 16.31212829107016660, 2.500000000000259348, 6.358241997069723261 ) ) ;
#2371=DIRECTION ( 'NONE',  ( 0.000000000000000000, 1.000000000000000000, 0.000000000000000000 ) ) ;
#2372=ADVANCED_FACE ( 'NONE', ( #1830 ), #63890, .T. ) ;
#2373=FACE_BOUND ( 'NONE', #69819, .T. ) ;
#2374=EDGE_LOOP ( 'NONE', ( #15043, #18988 ) ) ;
#2376=DIRECTION ( 'NONE',  ( 0.000000000000000000, 0.000000000000000000, 1.000000000000000000 ) ) ;
#2377=LINE ( 'NONE', #35108, #73188 ) ;
#2378=AXIS2_PLACEMENT_3D ( 'NONE', #85601, #25379, #46319 ) ;
#2380=AXIS2_PLACEMENT_3D ( 'NONE', #128646, #97221, #29145 ) ;
#2381=VECTOR ( 'NONE', #81570, 1000.000000000000000 ) ;
#2383=CARTESIAN_POINT ( 'NONE',  ( 15.83209681635531041, -1.500000000000000888, 5.404881881984402447 ) ) ;
#2385=DIRECTION ( 'NONE',  ( 0.000000000000000000, 0.000000000000000000, 1.000000000000000000 ) ) ;
#2386=CIRCLE ( 'NONE', #340, 0.1000000000000000472 ) ;
#2387=DIRECTION ( 'NONE',  ( 0.000000000000000000, 0.000000000000000000, -1.000000000000000000 ) ) ;
#2388=VERTEX_POINT ( 'NONE', #21480 ) ;
#2390=VECTOR ( 'NONE', #37748, 1000.000000000000000 ) ;
#2391=EDGE_LOOP ( 'NONE', ( #116054, #1797 ) ) ;
#2392=EDGE_LOOP ( 'NONE', ( #23017, #78011 ) ) ;
#2394=ORIENTED_EDGE ( 'NONE', *, *, #103651, .T. ) ;
#2395=VERTEX_POINT ( 'NONE', #41791 ) ;
#2396=CARTESIAN_POINT ( 'NONE',  ( -4.600000000000024514, 12.50000000000000000, 3.637306695894644726 ) ) ;
#2397=CARTESIAN_POINT ( 'NONE',  ( 4.599999999999940137, 2.500000000000000000, -4.230127018922201998 ) ) ;
#2398=EDGE_LOOP ( 'NONE', ( #19752, #25268 ) ) ;
#2399=FACE_BOUND ( 'NONE', #103410, .T. ) ;
#2400=PLANE ( 'NONE',  #95896 ) ;
#2401=EDGE_CURVE ( 'NONE', #77067, #110742, #80629, .T. ) ;
#2402=ORIENTED_EDGE ( 'NONE', *, *, #56485, .F. ) ;
#2403=CARTESIAN_POINT ( 'NONE',  ( 6.449999999999930012, 12.50000000000000000, 1.818653347947321475 ) ) ;
#2404=CARTESIAN_POINT ( 'NONE',  ( 9.149999999999916866, 2.500000000000000000, -1.472243186433550122 ) ) ;
#2405=DIRECTION ( 'NONE',  ( -0.000000000000000000, 1.000000000000000000, -0.000000000000000000 ) ) ;
#2407=CARTESIAN_POINT ( 'NONE',  ( 4.149999999999939959, 2.500000000000000000, -2.165063509461101710 ) ) ;
#2408=ADVANCED_FACE ( 'NONE', ( #39858 ), #76418, .T. ) ;
#2409=VERTEX_POINT ( 'NONE', #101339 ) ;
#2410=ORIENTED_EDGE ( 'NONE', *, *, #89206, .F. ) ;
#2411=VECTOR ( 'NONE', #32048, 1000.000000000000000 ) ;
#2412=ORIENTED_EDGE ( 'NONE', *, *, #86879, .T. ) ;
#2413=VECTOR ( 'NONE', #84929, 1000.000000000000000 ) ;
#2414=EDGE_CURVE ( 'NONE', #87409, #54592, #89576, .T. ) ;
#2415=FACE_OUTER_BOUND ( 'NONE', #71981, .T. ) ;
#2416=DIRECTION ( 'NONE',  ( 0.000000000000000000, -0.000000000000000000, 1.000000000000000000 ) ) ;
#2417=DIRECTION ( 'NONE',  ( 0.000000000000000000, 0.000000000000000000, 1.000000000000000000 ) ) ;
#2418=EDGE_CURVE ( 'NONE', #112557, #122705, #30679, .T. ) ;
#2419=ORIENTED_EDGE ( 'NONE', *, *, #15548, .F. ) ;
#2420=DIRECTION ( 'NONE',  ( 0.000000000000000000, 1.000000000000000000, 0.000000000000000000 ) ) ;
#2421=EDGE_CURVE ( 'NONE', #22876, #34089, #74353, .T. ) ;
#2422=FACE_OUTER_BOUND ( 'NONE', #55216, .T. ) ;
#2423=AXIS2_PLACEMENT_3D ( 'NONE', #23473, #91570, #101401 ) ;
#2424=CARTESIAN_POINT ( 'NONE',  ( 8.299999999999922551, 2.500000000000000000, -2.385244779468109755E-15 ) ) ;
#2425=AXIS2_PLACEMENT_3D ( 'NONE', #1646, #33076, #72979 ) ;
#2426=CARTESIAN_POINT ( 'NONE',  ( 10.64999999999990976, 12.50000000000000000, -6.148780366869526226 ) ) ;
#2427=EDGE_CURVE ( 'NONE', #29791, #85654, #34668, .T. ) ;
#2429=ORIENTED_EDGE ( 'NONE', *, *, #98433, .F. ) ;
#2430=AXIS2_PLACEMENT_3D ( 'NONE', #82803, #121412, #101140 ) ;
#2431=CARTESIAN_POINT ( 'NONE',  ( 2.049999999999950084, 12.50000000000000000, -6.430097255199264339 ) ) ;
#2432=VERTEX_POINT ( 'NONE', #111806 ) ;
#2433=CARTESIAN_POINT ( 'NONE',  ( 105.5000000000000142, 0.000000000000000000, 0.000000000000000000 ) ) ;
#2434=EDGE_CURVE ( 'NONE', #59088, #19851, #31668, .T. ) ;
#2435=CIRCLE ( 'NONE', #12894, 0.06509327318403745899 ) ;
#2436=EDGE_CURVE ( 'NONE', #93873, #74504, #75570, .T. ) ;
#2437=VERTEX_POINT ( 'NONE', #20840 ) ;
#2438=PLANE ( 'NONE',  #18318 ) ;
#2439=VERTEX_POINT ( 'NONE', #110502 ) ;
#2440=CARTESIAN_POINT ( 'NONE',  ( 1.049999999999952083, 12.50000000000000000, 6.841600689897072485 ) ) ;
#2441=DIRECTION ( 'NONE',  ( 0.000000000000000000, 0.000000000000000000, -1.000000000000000000 ) ) ;
#2442=FACE_OUTER_BOUND ( 'NONE', #24617, .T. ) ;
#2443=FACE_OUTER_BOUND ( 'NONE', #17284, .T. ) ;
#2445=ORIENTED_EDGE ( 'NONE', *, *, #104997, .F. ) ;
#2446=ORIENTED_EDGE ( 'NONE', *, *, #56336, .T. ) ;
#2447=CARTESIAN_POINT ( 'NONE',  ( -1.850000000000033840, 2.500000000000000000, 2.511473670974873507 ) ) ;
#2448=LINE ( 'NONE', #31941, #89179 ) ;
#2449=DIRECTION ( 'NONE',  ( 0.000000000000000000, 0.000000000000000000, -1.000000000000000000 ) ) ;
#2450=EDGE_LOOP ( 'NONE', ( #102947, #109387, #77285, #36067 ) ) ;
#2451=VERTEX_POINT ( 'NONE', #90198 ) ;
#2452=ORIENTED_EDGE ( 'NONE', *, *, #45661, .T. ) ;
#2453=DIRECTION ( 'NONE',  ( 0.000000000000000000, -0.000000000000000000, 1.000000000000000000 ) ) ;
#2454=CIRCLE ( 'NONE', #69266, 0.1000000000000002554 ) ;
#2455=VERTEX_POINT ( 'NONE', #2463 ) ;
#2456=FACE_OUTER_BOUND ( 'NONE', #93514, .T. ) ;
#2457=DIRECTION ( 'NONE',  ( 0.000000000000000000, 1.000000000000000000, 0.000000000000000000 ) ) ;
#2458=CIRCLE ( 'NONE', #90281, 0.09999999999999999167 ) ;
#2459=DIRECTION ( 'NONE',  ( 0.000000000000000000, 0.000000000000000000, -1.000000000000000000 ) ) ;
#2460=EDGE_LOOP ( 'NONE', ( #6522, #89055 ) ) ;
#2461=CARTESIAN_POINT ( 'NONE',  ( 5.199999999999933564, 2.500000000000000000, 0.4464101615137735513 ) ) ;
#2462=CARTESIAN_POINT ( 'NONE',  ( 6.249999999999932498, 2.500000000000000000, 5.902370205355745192 ) ) ;
#2463=CARTESIAN_POINT ( 'NONE',  ( 7.699999999999925571, 2.500000000000000000, -4.576537180435978236 ) ) ;
#2464=PLANE ( 'NONE',  #59350 ) ;
#2465=FACE_OUTER_BOUND ( 'NONE', #114572, .T. ) ;
#2466=ORIENTED_EDGE ( 'NONE', *, *, #47546, .T. ) ;
#2467=CONICAL_SURFACE ( 'NONE', #77772, 0.1000000000000002554, 0.003490658503988666988 ) ;
#2468=AXIS2_PLACEMENT_3D ( 'NONE', #105545, #6032, #68176 ) ;
#2469=CARTESIAN_POINT ( 'NONE',  ( -7.500000000000011546, 2.500000000000000000, 3.537306695894645081 ) ) ;
#2470=AXIS2_PLACEMENT_3D ( 'NONE', #85895, #113601, #86551 ) ;
#2471=VECTOR ( 'NONE', #96940, 1000.000000000000000 ) ;
#2472=CARTESIAN_POINT ( 'NONE',  ( 65.34954526970105348, -3.515384427006628787, 5.621991122703798638 ) ) ;
#2473=EDGE_LOOP ( 'NONE', ( #36913, #54590, #21796, #46091 ) ) ;
#2474=ORIENTED_EDGE ( 'NONE', *, *, #116064, .T. ) ;
#2476=LINE ( 'NONE', #121613, #124283 ) ;
#2477=CARTESIAN_POINT ( 'NONE',  ( -11.84999999999999609, 2.500000000000000000, 6.741600689897071952 ) ) ;
#2478=CIRCLE ( 'NONE', #71431, 0.1000000000000002554 ) ;
#2479=LINE ( 'NONE', #53543, #94922 ) ;
#2480=FACE_OUTER_BOUND ( 'NONE', #114483, .T. ) ;
#2481=VECTOR ( 'NONE', #88524, 1000.000000000000000 ) ;
#2482=EDGE_CURVE ( 'NONE', #85597, #54227, #117303, .T. ) ;
#2483=DIRECTION ( 'NONE',  ( 0.000000000000000000, 0.000000000000000000, 1.000000000000000000 ) ) ;
#2484=VECTOR ( 'NONE', #17187, 1000.000000000000000 ) ;
#2485=CARTESIAN_POINT ( 'NONE',  ( 12.94999999999989981, 2.500000000000000000, -2.065063509461102065 ) ) ;
#2486=FACE_OUTER_BOUND ( 'NONE', #113369, .T. ) ;
#2487=CONICAL_SURFACE ( 'NONE', #42519, 0.1000000000000002554, 0.003490658503988666988 ) ;
#2488=AXIS2_PLACEMENT_3D ( 'NONE', #93850, #116540, #113480 ) ;
#2489=CARTESIAN_POINT ( 'NONE',  ( -2.499999999999996447, 2.500000000000000000, 4.430127018922196847 ) ) ;
#2490=ORIENTED_EDGE ( 'NONE', *, *, #78998, .T. ) ;
#2491=EDGE_LOOP ( 'NONE', ( #88964, #44101 ) ) ;
#2492=VERTEX_POINT ( 'NONE', #90863 ) ;
#2493=EDGE_LOOP ( 'NONE', ( #84936, #36789 ) ) ;
#2494=LINE ( 'NONE', #79786, #16919 ) ;
#2495=CARTESIAN_POINT ( 'NONE',  ( -15.19999999999998330, 2.500000000000000000, 0.3464101615137758494 ) ) ;
#2496=ORIENTED_EDGE ( 'NONE', *, *, #72490, .F. ) ;
#2497=FACE_OUTER_BOUND ( 'NONE', #36409, .T. ) ;
#2498=LINE ( 'NONE', #1869, #5132 ) ;
#2499=CARTESIAN_POINT ( 'NONE',  ( -0.6500000000000403233, 12.50000000000000000, 6.148780366869520009 ) ) ;
#2500=VERTEX_POINT ( 'NONE', #49674 ) ;
#2501=LINE ( 'NONE', #72570, #7631 ) ;
#2502=CARTESIAN_POINT ( 'NONE',  ( 9.199999999999915801, 2.500000000000000000, 4.330127018922196314 ) ) ;
#2503=EDGE_LOOP ( 'NONE', ( #104639, #31206 ) ) ;
#2504=ORIENTED_EDGE ( 'NONE', *, *, #51530, .F. ) ;
#2505=VERTEX_POINT ( 'NONE', #72529 ) ;
#2506=AXIS2_PLACEMENT_3D ( 'NONE', #113004, #44253, #4968 ) ;
#2507=ORIENTED_EDGE ( 'NONE', *, *, #12285, .T. ) ;
#2508=DIRECTION ( 'NONE',  ( -0.000000000000000000, 1.000000000000000000, -0.000000000000000000 ) ) ;
#2509=CONICAL_SURFACE ( 'NONE', #46438, 0.09999999999999982514, 0.003490658503988666988 ) ;
#2510=CONICAL_SURFACE ( 'NONE', #4645, 0.1000000000000000472, 0.003490658503988666988 ) ;
#2511=CARTESIAN_POINT ( 'NONE',  ( 6.849999999999929479, 2.500000000000000000, 6.148780366869520009 ) ) ;
#2512=CARTESIAN_POINT ( 'NONE',  ( 5.849999999999932143, 12.50000000000000000, 2.165063509461097713 ) ) ;
#2513=CARTESIAN_POINT ( 'NONE',  ( -6.450000000000014388, 12.50000000000000000, 1.883746621131358934 ) ) ;
#2514=EDGE_CURVE ( 'NONE', #38961, #26037, #31321, .T. ) ;
#2515=CIRCLE ( 'NONE', #69426, 0.1000000000000002554 ) ;
#2516=ORIENTED_EDGE ( 'NONE', *, *, #90834, .F. ) ;
#2517=AXIS2_PLACEMENT_3D ( 'NONE', #83803, #33441, #44527 ) ;
#2518=DIRECTION ( 'NONE',  ( -4.274815082592931898E-19, -0.9999939076577903929, -0.003490651415223739937 ) ) ;
#2519=CIRCLE ( 'NONE', #44399, 0.09999999999999999167 ) ;
#2520=ORIENTED_EDGE ( 'NONE', *, *, #53103, .F. ) ;
#2521=DIRECTION ( 'NONE',  ( 0.000000000000000000, -0.9999939076577903929, 0.003490651415223739937 ) ) ;
#2522=CARTESIAN_POINT ( 'NONE',  ( -6.650000000000019007, 2.500000000000000000, -1.572243186433550211 ) ) ;
#2524=DIRECTION ( 'NONE',  ( 0.000000000000000000, 1.000000000000000000, 0.000000000000000000 ) ) ;
#2525=DIRECTION ( 'NONE',  ( -0.000000000000000000, -1.000000000000000000, -0.000000000000000000 ) ) ;
#2526=EDGE_CURVE ( 'NONE', #83361, #34821, #16953, .T. ) ;
#2527=VECTOR ( 'NONE', #43741, 1000.000000000000000 ) ;
#2528=ORIENTED_EDGE ( 'NONE', *, *, #46934, .T. ) ;
#2529=EDGE_LOOP ( 'NONE', ( #120920, #38975, #4099, #127621 ) ) ;
#2530=EDGE_CURVE ( 'NONE', #112123, #66032, #90130, .T. ) ;
#2531=ADVANCED_FACE ( 'NONE', ( #124841 ), #62960, .T. ) ;
#2532=ORIENTED_EDGE ( 'NONE', *, *, #65929, .T. ) ;
#2533=CARTESIAN_POINT ( 'NONE',  ( -3.350000000000031619, 12.50000000000000000, -5.867463478539787225 ) ) ;
#2534=DIRECTION ( 'NONE',  ( 0.000000000000000000, 1.000000000000000000, 0.000000000000000000 ) ) ;
#2535=CARTESIAN_POINT ( 'NONE',  ( 3.349999999999945466, 2.500000000000000000, -2.957883832488653830 ) ) ;
#2536=ADVANCED_FACE ( 'NONE', ( #74450 ), #60907, .T. ) ;
#2537=FACE_BOUND ( 'NONE', #110485, .T. ) ;
#2538=DIRECTION ( 'NONE',  ( 0.000000000000000000, 1.000000000000000000, 0.000000000000000000 ) ) ;
#2539=CARTESIAN_POINT ( 'NONE',  ( 11.89999999999990443, 2.500000000000000000, -0.4464101615137782142 ) ) ;
#2540=DIRECTION ( 'NONE',  ( -0.000000000000000000, -1.000000000000000000, -0.000000000000000000 ) ) ;
#2541=CARTESIAN_POINT ( 'NONE',  ( -5.850000000000021849, 2.500000000000000000, -2.957883832488653830 ) ) ;
#2542=DIRECTION ( 'NONE',  ( 0.000000000000000000, -0.000000000000000000, 1.000000000000000000 ) ) ;
#2543=CARTESIAN_POINT ( 'NONE',  ( -0.6000000000000323963, 2.500000000000000000, -0.4464101615137759382 ) ) ;
#2544=VERTEX_POINT ( 'NONE', #12924 ) ;
#2545=DIRECTION ( 'NONE',  ( -0.000000000000000000, -1.000000000000000000, -0.000000000000000000 ) ) ;
#2546=CARTESIAN_POINT ( 'NONE',  ( -4.350000000000027178, 2.500000000000000000, -6.841600689897077814 ) ) ;
#2547=ORIENTED_EDGE ( 'NONE', *, *, #57080, .T. ) ;
#2548=ORIENTED_EDGE ( 'NONE', *, *, #18075, .T. ) ;
#2549=DIRECTION ( 'NONE',  ( 0.000000000000000000, 0.000000000000000000, -1.000000000000000000 ) ) ;
#2550=DIRECTION ( 'NONE',  ( -0.000000000000000000, -1.000000000000000000, -0.000000000000000000 ) ) ;
#2551=FACE_BOUND ( 'NONE', #118144, .T. ) ;
#2552=LINE ( 'NONE', #82451, #28539 ) ;
#2553=AXIS2_PLACEMENT_3D ( 'NONE', #111461, #83928, #125161 ) ;
#2554=CIRCLE ( 'NONE', #42390, 0.06509327318403745899 ) ;
#2555=CIRCLE ( 'NONE', #117464, 0.1000000000000002554 ) ;
#2556=ORIENTED_EDGE ( 'NONE', *, *, #10699, .T. ) ;
#2557=FACE_OUTER_BOUND ( 'NONE', #56731, .T. ) ;
#2558=DIRECTION ( 'NONE',  ( 0.000000000000000000, 1.000000000000000000, 0.000000000000000000 ) ) ;
#2559=ORIENTED_EDGE ( 'NONE', *, *, #47085, .T. ) ;
#2560=AXIS2_PLACEMENT_3D ( 'NONE', #69678, #19944, #6860 ) ;
#2561=DIRECTION ( 'NONE',  ( 0.000000000000000000, 1.000000000000000000, 0.000000000000000000 ) ) ;
#2562=CARTESIAN_POINT ( 'NONE',  ( 11.84999999999990372, 12.50000000000000000, 1.818653347947321475 ) ) ;
#2563=CIRCLE ( 'NONE', #50610, 0.1000000000000002554 ) ;
#2564=AXIS2_PLACEMENT_3D ( 'NONE', #92964, #53670, #123676 ) ;
#2565=AXIS2_PLACEMENT_3D ( 'NONE', #81835, #21647, #29534 ) ;
#2566=AXIS2_PLACEMENT_3D ( 'NONE', #66194, #115268, #6596 ) ;
#2567=EDGE_CURVE ( 'NONE', #26449, #109816, #10706, .T. ) ;
#2568=VERTEX_POINT ( 'NONE', #53528 ) ;
#2569=EDGE_CURVE ( 'NONE', #21611, #86863, #21196, .T. ) ;
#2570=DIRECTION ( 'NONE',  ( 0.000000000000000000, 1.000000000000000000, 0.000000000000000000 ) ) ;
#2571=DIRECTION ( 'NONE',  ( 0.000000000000000000, 1.000000000000000000, 0.000000000000000000 ) ) ;
#2572=AXIS2_PLACEMENT_3D ( 'NONE', #24465, #114131, #64381 ) ;
#2573=ADVANCED_FACE ( 'NONE', ( #14847 ), #106860, .T. ) ;
#2574=ORIENTED_EDGE ( 'NONE', *, *, #9119, .T. ) ;
#2575=CARTESIAN_POINT ( 'NONE',  ( -2.700000000000029932, 2.500000000000000000, -0.4464101615137782142 ) ) ;
#2576=CIRCLE ( 'NONE', #19310, 0.1000000000000000472 ) ;
#2578=CARTESIAN_POINT ( 'NONE',  ( 2.699999999999945555, 2.500000000000000000, 4.083716857408420609 ) ) ;
#2579=ADVANCED_FACE ( 'NONE', ( #83633 ), #112452, .T. ) ;
#2580=VERTEX_POINT ( 'NONE', #104550 ) ;
#2581=VERTEX_POINT ( 'NONE', #93443 ) ;
#2582=EDGE_CURVE ( 'NONE', #37773, #72985, #94344, .T. ) ;
#2583=PLANE ( 'NONE',  #65990 ) ;
#2584=EDGE_CURVE ( 'NONE', #55889, #77376, #123592, .T. ) ;
#2585=EDGE_LOOP ( 'NONE', ( #117318, #4173 ) ) ;
#2586=DIRECTION ( 'NONE',  ( 0.000000000000000000, 1.000000000000000000, 0.000000000000000000 ) ) ;
#2587=CARTESIAN_POINT ( 'NONE',  ( 9.399999999999915090, 12.50000000000000000, 3.918623584224383727 ) ) ;
#2588=EDGE_CURVE ( 'NONE', #54197, #54180, #19117, .T. ) ;
#2589=EDGE_CURVE ( 'NONE', #44930, #83361, #84907, .T. ) ;
#2590=CARTESIAN_POINT ( 'NONE',  ( 7.499999999999960032, 2.500000000000000000, -0.1000000000000022815 ) ) ;
#2591=ORIENTED_EDGE ( 'NONE', *, *, #117354, .T. ) ;
#2592=DIRECTION ( 'NONE',  ( -0.000000000000000000, 1.000000000000000000, -0.000000000000000000 ) ) ;
#2593=DIRECTION ( 'NONE',  ( -0.000000000000000000, 1.000000000000000000, -0.000000000000000000 ) ) ;
#2594=CARTESIAN_POINT ( 'NONE',  ( 5.399999999999936406, 2.500000000000000000, -3.637306695894650055 ) ) ;
#2595=FACE_OUTER_BOUND ( 'NONE', #126876, .T. ) ;
#2596=DIRECTION ( 'NONE',  ( -0.000000000000000000, -1.000000000000000000, -0.000000000000000000 ) ) ;
#2597=AXIS2_PLACEMENT_3D ( 'NONE', #8601, #106812, #36813 ) ;
#2598=DIRECTION ( 'NONE',  ( 0.000000000000000000, 1.000000000000000000, 0.000000000000000000 ) ) ;
#2599=EDGE_CURVE ( 'NONE', #16102, #105827, #127805, .T. ) ;
#2600=ORIENTED_EDGE ( 'NONE', *, *, #82184, .T. ) ;
#2601=VERTEX_POINT ( 'NONE', #82996 ) ;
#2602=CARTESIAN_POINT ( 'NONE',  ( 6.249999999999932498, 2.500000000000000000, -2.957883832488653830 ) ) ;
#2603=ORIENTED_EDGE ( 'NONE', *, *, #113504, .F. ) ;
#2604=AXIS2_PLACEMENT_3D ( 'NONE', #11427, #99823, #110274 ) ;
#2605=LINE ( 'NONE', #53021, #68153 ) ;
#2606=AXIS2_PLACEMENT_3D ( 'NONE', #81180, #73931, #113864 ) ;
#2607=VECTOR ( 'NONE', #26167, 1000.000000000000000 ) ;
#2608=ORIENTED_EDGE ( 'NONE', *, *, #38797, .F. ) ;
#2609=ORIENTED_EDGE ( 'NONE', *, *, #41208, .F. ) ;
#2610=ORIENTED_EDGE ( 'NONE', *, *, #58219, .T. ) ;
#2611=CARTESIAN_POINT ( 'NONE',  ( -9.600000000000008527, 2.500000000000000000, -5.122947341949750211 ) ) ;
#2612=FACE_OUTER_BOUND ( 'NONE', #65621, .T. ) ;
#2613=CIRCLE ( 'NONE', #92508, 0.06509327318403745899 ) ;
#2614=AXIS2_PLACEMENT_3D ( 'NONE', #80446, #120370, #128922 ) ;
#2615=DIRECTION ( 'NONE',  ( -0.000000000000000000, 1.000000000000000000, -0.000000000000000000 ) ) ;
#2616=CONICAL_SURFACE ( 'NONE', #59073, 0.09999999999999982514, 0.003490658503988666988 ) ;
#2617=CARTESIAN_POINT ( 'NONE',  ( 6.249999999999965361, 2.500000000000000000, 2.265063509461097357 ) ) ;
#2618=FACE_OUTER_BOUND ( 'NONE', #124727, .T. ) ;
#2619=CARTESIAN_POINT ( 'NONE',  ( 1.649999999999951505, 2.500000000000000000, 2.957883832488649389 ) ) ;
#2620=DIRECTION ( 'NONE',  ( 0.000000000000000000, 0.000000000000000000, 1.000000000000000000 ) ) ;
#2621=CARTESIAN_POINT ( 'NONE',  ( 7.499999999999925393, 2.500000000000000000, 5.022947341949748790 ) ) ;
#2622=CARTESIAN_POINT ( 'NONE',  ( 6.449999999999930012, 2.500000000000000000, -1.718653347947326049 ) ) ;
#2623=AXIS2_PLACEMENT_3D ( 'NONE', #10238, #77044, #116945 ) ;
#2624=ORIENTED_EDGE ( 'NONE', *, *, #76613, .F. ) ;
#2625=CARTESIAN_POINT ( 'NONE',  ( 3.949999999999941558, 2.500000000000000000, -6.048780366869526581 ) ) ;
#2626=ORIENTED_EDGE ( 'NONE', *, *, #109397, .F. ) ;
#2627=VERTEX_POINT ( 'NONE', #95378 ) ;
#2628=DIRECTION ( 'NONE',  ( -0.000000000000000000, -1.000000000000000000, -0.000000000000000000 ) ) ;
#2629=DIRECTION ( 'NONE',  ( 0.000000000000000000, 0.000000000000000000, 1.000000000000000000 ) ) ;
#2630=DIRECTION ( 'NONE',  ( 0.000000000000000000, 0.000000000000000000, -1.000000000000000000 ) ) ;
#2631=CIRCLE ( 'NONE', #105042, 0.06509327318403745899 ) ;
#2632=CARTESIAN_POINT ( 'NONE',  ( 8.949999999999915801, 2.500000000000000000, 6.841600689897072485 ) ) ;
#2633=EDGE_CURVE ( 'NONE', #111448, #113894, #121532, .T. ) ;
#2634=DIRECTION ( 'NONE',  ( 0.000000000000000000, 0.000000000000000000, 1.000000000000000000 ) ) ;
#2636=FACE_OUTER_BOUND ( 'NONE', #91479, .T. ) ;
#2637=ORIENTED_EDGE ( 'NONE', *, *, #71743, .F. ) ;
#2638=AXIS2_PLACEMENT_3D ( 'NONE', #126653, #95261, #38275 ) ;
#2639=CIRCLE ( 'NONE', #107205, 0.06509327318403745899 ) ;
#2640=ORIENTED_EDGE ( 'NONE', *, *, #36405, .F. ) ;
#2641=CONICAL_SURFACE ( 'NONE', #61154, 0.1000000000000002554, 0.003490658503988666988 ) ;
#2642=ORIENTED_EDGE ( 'NONE', *, *, #1850, .T. ) ;
#2643=ORIENTED_EDGE ( 'NONE', *, *, #126696, .T. ) ;
#2644=EDGE_CURVE ( 'NONE', #113, #119313, #85550, .T. ) ;
#2645=ORIENTED_EDGE ( 'NONE', *, *, #84372, .T. ) ;
#2646=CIRCLE ( 'NONE', #600, 0.1000000000000002554 ) ;
#2647=CARTESIAN_POINT ( 'NONE',  ( -8.300000000000009592, 2.500000000000000000, 4.330127018922196314 ) ) ;
#2648=LINE ( 'NONE', #103456, #31041 ) ;
#2649=VECTOR ( 'NONE', #42428, 1000.000000000000000 ) ;
#2650=AXIS2_PLACEMENT_3D ( 'NONE', #59785, #20485, #51249 ) ;
#2651=LINE ( 'NONE', #32798, #100813 ) ;
#2652=DIRECTION ( 'NONE',  ( 0.000000000000000000, 1.000000000000000000, 0.000000000000000000 ) ) ;
#2653=DIRECTION ( 'NONE',  ( 0.000000000000000000, -0.9999939076577903929, 0.003490651415223739937 ) ) ;
#2654=VERTEX_POINT ( 'NONE', #35811 ) ;
#2655=DIRECTION ( 'NONE',  ( 0.000000000000000000, 0.000000000000000000, -1.000000000000000000 ) ) ;
#2656=DIRECTION ( 'NONE',  ( 0.000000000000000000, 0.000000000000000000, 1.000000000000000000 ) ) ;
#2657=DIRECTION ( 'NONE',  ( 0.000000000000000000, 0.000000000000000000, 1.000000000000000000 ) ) ;
#2658=CIRCLE ( 'NONE', #10970, 0.1000000000000002554 ) ;
#2659=CONICAL_SURFACE ( 'NONE', #17225, 0.1000000000000002554, 0.003490658503988666988 ) ;
#2660=DIRECTION ( 'NONE',  ( 0.000000000000000000, 1.000000000000000000, 0.000000000000000000 ) ) ;
#2661=ORIENTED_EDGE ( 'NONE', *, *, #5829, .F. ) ;
#2662=VECTOR ( 'NONE', #122271, 1000.000000000000000 ) ;
#2663=CONICAL_SURFACE ( 'NONE', #27806, 0.09999999999999982514, 0.003490658503988666988 ) ;
#2664=CONICAL_SURFACE ( 'NONE', #56944, 0.1000000000000002554, 0.003490658503988666988 ) ;
#2665=ORIENTED_EDGE ( 'NONE', *, *, #76878, .T. ) ;
#2666=ORIENTED_EDGE ( 'NONE', *, *, #6673, .T. ) ;
#2667=DIRECTION ( 'NONE',  ( 0.000000000000000000, 0.000000000000000000, 1.000000000000000000 ) ) ;
#2668=CIRCLE ( 'NONE', #15186, 0.06509327318403745899 ) ;
#2669=VERTEX_POINT ( 'NONE', #52879 ) ;
#2670=DIRECTION ( 'NONE',  ( -0.000000000000000000, 1.000000000000000000, -0.000000000000000000 ) ) ;
#2671=DIRECTION ( 'NONE',  ( 0.000000000000000000, 1.000000000000000000, 0.000000000000000000 ) ) ;
#2672=ADVANCED_FACE ( 'NONE', ( #24064 ), #103910, .T. ) ;
#2673=AXIS2_PLACEMENT_3D ( 'NONE', #118990, #108523, #9683 ) ;
#2674=EDGE_LOOP ( 'NONE', ( #118146, #2120, #127648, #44713 ) ) ;
#2675=CARTESIAN_POINT ( 'NONE',  ( 4.149999999999938183, 2.500000000000000000, 7.188010851410848723 ) ) ;
#2676=CARTESIAN_POINT ( 'NONE',  ( -0.8000000000000315747, 2.500000000000000000, 0.000000000000000000 ) ) ;
#2678=FACE_OUTER_BOUND ( 'NONE', #23150, .T. ) ;
#2679=EDGE_CURVE ( 'NONE', #40817, #112302, #37925, .T. ) ;
#2680=DIRECTION ( 'NONE',  ( -0.000000000000000000, -1.000000000000000000, -0.000000000000000000 ) ) ;
#2681=ORIENTED_EDGE ( 'NONE', *, *, #7492, .F. ) ;
#2682=EDGE_CURVE ( 'NONE', #50283, #18676, #54636, .T. ) ;
#2683=ADVANCED_FACE ( 'NONE', ( #67842 ), #47574, .T. ) ;
#2684=AXIS2_PLACEMENT_3D ( 'NONE', #25158, #123368, #77971 ) ;
#2685=EDGE_LOOP ( 'NONE', ( #117186, #55891, #76035, #100290 ) ) ;
#2686=VECTOR ( 'NONE', #45189, 1000.000000000000000 ) ;
#2687=EDGE_CURVE ( 'NONE', #81254, #110135, #46938, .T. ) ;
#2689=ADVANCED_FACE ( 'NONE', ( #97946 ), #67167, .T. ) ;
#2690=EDGE_CURVE ( 'NONE', #11740, #104068, #71359, .T. ) ;
#2691=CARTESIAN_POINT ( 'NONE',  ( 7.949999999999925571, 2.500000000000000000, -6.495190528383302464 ) ) ;
#2692=CARTESIAN_POINT ( 'NONE',  ( -7.500000000000013323, 12.50000000000000000, 5.022947341949748790 ) ) ;
#2693=CARTESIAN_POINT ( 'NONE',  ( -8.950000000000009948, 12.50000000000000000, -1.818653347947326138 ) ) ;
#2694=ORIENTED_EDGE ( 'NONE', *, *, #15092, .T. ) ;
#2695=AXIS2_PLACEMENT_3D ( 'NONE', #88821, #128777, #39108 ) ;
#2696=VECTOR ( 'NONE', #41880, 1000.000000000000000 ) ;
#2697=CONICAL_SURFACE ( 'NONE', #126034, 0.09999999999999982514, 0.003490658503988666988 ) ;
#2698=CIRCLE ( 'NONE', #63365, 0.1000000000000002554 ) ;
#2699=EDGE_LOOP ( 'NONE', ( #114872, #20001 ) ) ;
#2700=DIRECTION ( 'NONE',  ( 0.000000000000000000, 0.000000000000000000, 1.000000000000000000 ) ) ;
#2701=DIRECTION ( 'NONE',  ( 0.000000000000000000, 0.000000000000000000, 1.000000000000000000 ) ) ;
#2702=EDGE_CURVE ( 'NONE', #34419, #6486, #88066, .T. ) ;
#2703=DIRECTION ( 'NONE',  ( 0.000000000000000000, 0.000000000000000000, 1.000000000000000000 ) ) ;
#2704=CARTESIAN_POINT ( 'NONE',  ( 4.999999999999973355, 2.500000000000000000, -4.330127018922201643 ) ) ;
#2705=ORIENTED_EDGE ( 'NONE', *, *, #116804, .T. ) ;
#2706=EDGE_CURVE ( 'NONE', #72427, #46092, #81828, .T. ) ;
#2708=CARTESIAN_POINT ( 'NONE',  ( -3.350000000000028955, 2.500000000000000000, 5.802370205355744659 ) ) ;
#2709=EDGE_CURVE ( 'NONE', #34681, #94526, #127417, .T. ) ;
#2710=AXIS2_PLACEMENT_3D ( 'NONE', #39092, #68517, #18775 ) ;
#2712=CARTESIAN_POINT ( 'NONE',  ( -1.050000000000038236, 2.500000000000000000, -1.918653347947326004 ) ) ;
#2713=AXIS2_PLACEMENT_3D ( 'NONE', #122251, #3116, #91484 ) ;
#2715=AXIS2_PLACEMENT_3D ( 'NONE', #49441, #89349, #99819 ) ;
#2716=CARTESIAN_POINT ( 'NONE',  ( 8.749999999999957367, 12.50000000000000000, 2.099970236277060032 ) ) ;
#2717=ORIENTED_EDGE ( 'NONE', *, *, #67235, .T. ) ;
#2718=AXIS2_PLACEMENT_3D ( 'NONE', #41013, #80915, #120835 ) ;
#2719=DIRECTION ( 'NONE',  ( 0.000000000000000000, 0.000000000000000000, 1.000000000000000000 ) ) ;
#2720=EDGE_LOOP ( 'NONE', ( #9302, #35012 ) ) ;
#2721=LINE ( 'NONE', #62939, #86192 ) ;
#2722=FACE_OUTER_BOUND ( 'NONE', #5768, .T. ) ;
#2723=ORIENTED_EDGE ( 'NONE', *, *, #70197, .T. ) ;
#2724=EDGE_LOOP ( 'NONE', ( #70477, #76376, #25055, #26694 ) ) ;
#2725=LINE ( 'NONE', #101587, #58190 ) ;
#2726=CARTESIAN_POINT ( 'NONE',  ( -3.100000000000028511, 2.500000000000000000, -4.776537180435977525 ) ) ;
#2727=AXIS2_PLACEMENT_3D ( 'NONE', #25087, #14602, #92533 ) ;
#2730=CARTESIAN_POINT ( 'NONE',  ( -10.85000000000000142, 2.500000000000000000, -6.495190528383298911 ) ) ;
#2731=DIRECTION ( 'NONE',  ( 0.000000000000000000, 0.000000000000000000, 1.000000000000000000 ) ) ;
#2732=DIRECTION ( 'NONE',  ( 0.000000000000000000, -0.000000000000000000, 1.000000000000000000 ) ) ;
#2733=CARTESIAN_POINT ( 'NONE',  ( -2.900000000000029221, 12.50000000000000000, -0.6928203230275541413 ) ) ;
#2734=CARTESIAN_POINT ( 'NONE',  ( -3.950000000000029932, 2.500000000000000000, -6.048780366869526581 ) ) ;
#2735=AXIS2_PLACEMENT_3D ( 'NONE', #53251, #12017, #94440 ) ;
#2736=ADVANCED_FACE ( 'NONE', ( #106483 ), #42133, .T. ) ;
#2737=CONICAL_SURFACE ( 'NONE', #29951, 0.1000000000000002554, 0.003490658503988666988 ) ;
#2738=CIRCLE ( 'NONE', #75908, 0.09999999999999982514 ) ;
#2739=ORIENTED_EDGE ( 'NONE', *, *, #111630, .F. ) ;
#2740=ADVANCED_FACE ( 'NONE', ( #27922 ), #86835, .T. ) ;
#2741=EDGE_LOOP ( 'NONE', ( #15690, #56889, #85690, #21277 ) ) ;
#2742=DIRECTION ( 'NONE',  ( 0.000000000000000000, -0.9999939076577903929, 0.003490651415223739937 ) ) ;
#2743=ORIENTED_EDGE ( 'NONE', *, *, #22817, .F. ) ;
#2744=LINE ( 'NONE', #112070, #122776 ) ;
#2745=CARTESIAN_POINT ( 'NONE',  ( -11.84999999999999609, 2.500000000000000000, 6.048780366869521252 ) ) ;
#2746=CARTESIAN_POINT ( 'NONE',  ( -6.050000000000022027, 12.50000000000000000, -1.818653347947326138 ) ) ;
#2747=ORIENTED_EDGE ( 'NONE', *, *, #127482, .F. ) ;
#2748=EDGE_LOOP ( 'NONE', ( #74714, #97201 ) ) ;
#2749=FACE_BOUND ( 'NONE', #15038, .T. ) ;
#2751=ADVANCED_FACE ( 'NONE', ( #118234 ), #88100, .T. ) ;
#2752=AXIS2_PLACEMENT_3D ( 'NONE', #113963, #23646, #83844 ) ;
#2753=DIRECTION ( 'NONE',  ( -0.000000000000000000, 1.000000000000000000, -0.000000000000000000 ) ) ;
#2754=CARTESIAN_POINT ( 'NONE',  ( 17.79089025268843827, -2.511997385349134415, 2.795007471442847002 ) ) ;
#2755=VECTOR ( 'NONE', #54178, 1000.000000000000000 ) ;
#2756=EDGE_CURVE ( 'NONE', #60318, #53692, #16783, .T. ) ;
#2757=CIRCLE ( 'NONE', #90483, 0.06509327318403745899 ) ;
#2758=DIRECTION ( 'NONE',  ( 0.000000000000000000, 1.000000000000000000, 0.000000000000000000 ) ) ;
#2759=DIRECTION ( 'NONE',  ( -0.000000000000000000, 1.000000000000000000, -0.000000000000000000 ) ) ;
#2760=CONICAL_SURFACE ( 'NONE', #11062, 0.1000000000000002554, 0.003490658503988666988 ) ;
#2761=CARTESIAN_POINT ( 'NONE',  ( -11.84999999999999787, 2.500000000000000000, -6.841600689897074261 ) ) ;
#2763=DIRECTION ( 'NONE',  ( 0.000000000000000000, 1.000000000000000000, 0.000000000000000000 ) ) ;
#2764=CARTESIAN_POINT ( 'NONE',  ( 2.899999999999946620, 2.500000000000000000, -0.6928203230275542523 ) ) ;
#2765=DIRECTION ( 'NONE',  ( 0.000000000000000000, 1.000000000000000000, 0.000000000000000000 ) ) ;
#2766=DIRECTION ( 'NONE',  ( 0.000000000000000000, 1.000000000000000000, 0.000000000000000000 ) ) ;
#2767=DIRECTION ( 'NONE',  ( 0.000000000000000000, 0.000000000000000000, -1.000000000000000000 ) ) ;
#2768=AXIS2_PLACEMENT_3D ( 'NONE', #116367, #45078, #5754 ) ;
#2769=LINE ( 'NONE', #838, #101550 ) ;
#2770=EDGE_CURVE ( 'NONE', #78466, #109968, #58678, .T. ) ;
#2771=EDGE_LOOP ( 'NONE', ( #86641, #125935 ) ) ;
#2772=ORIENTED_EDGE ( 'NONE', *, *, #76296, .T. ) ;
#2773=ORIENTED_EDGE ( 'NONE', *, *, #42941, .F. ) ;
#2774=DIRECTION ( 'NONE',  ( 0.000000000000000000, 0.000000000000000000, -1.000000000000000000 ) ) ;
#2775=AXIS2_PLACEMENT_3D ( 'NONE', #21221, #71612, #12045 ) ;
#2776=ORIENTED_EDGE ( 'NONE', *, *, #84116, .T. ) ;
#2777=AXIS2_PLACEMENT_3D ( 'NONE', #7477, #30371, #38251 ) ;
#2778=AXIS2_PLACEMENT_3D ( 'NONE', #73139, #30652, #20818 ) ;
#2779=CARTESIAN_POINT ( 'NONE',  ( 11.64999999999990443, 2.500000000000000000, -5.702370205355749455 ) ) ;
#2780=ORIENTED_EDGE ( 'NONE', *, *, #6961, .T. ) ;
#2781=EDGE_LOOP ( 'NONE', ( #104980, #33286, #114242, #8049 ) ) ;
#2782=VERTEX_POINT ( 'NONE', #128734 ) ;
#2783=VECTOR ( 'NONE', #25937, 1000.000000000000000 ) ;
#2784=CARTESIAN_POINT ( 'NONE',  ( 3.949999999999942446, 2.500000000000000000, -6.941600689897078347 ) ) ;
#2785=FACE_OUTER_BOUND ( 'NONE', #35121, .T. ) ;
#2786=AXIS2_PLACEMENT_3D ( 'NONE', #75674, #122866, #103222 ) ;
#2787=DIRECTION ( 'NONE',  ( -0.000000000000000000, 1.000000000000000000, -0.000000000000000000 ) ) ;
#2788=CARTESIAN_POINT ( 'NONE',  ( -7.100000000000017408, 12.50000000000000000, 0.6277270498435120194 ) ) ;
#2789=CARTESIAN_POINT ( 'NONE',  ( 3.549999999999944755, 12.50000000000000000, -6.776507416713039689 ) ) ;
#2790=DIRECTION ( 'NONE',  ( -0.000000000000000000, 1.000000000000000000, -0.000000000000000000 ) ) ;
#2791=ADVANCED_FACE ( 'NONE', ( #75722 ), #116286, .T. ) ;
#2792=ORIENTED_EDGE ( 'NONE', *, *, #117683, .F. ) ;
#2793=DIRECTION ( 'NONE',  ( 0.000000000000000000, 0.000000000000000000, 1.000000000000000000 ) ) ;
#2794=VERTEX_POINT ( 'NONE', #57387 ) ;
#2795=ORIENTED_EDGE ( 'NONE', *, *, #95965, .F. ) ;
#2796=ORIENTED_EDGE ( 'NONE', *, *, #29487, .F. ) ;
#2797=EDGE_CURVE ( 'NONE', #44668, #51310, #23245, .T. ) ;
#2799=AXIS2_PLACEMENT_3D ( 'NONE', #118385, #8423, #18252 ) ;
#2800=CIRCLE ( 'NONE', #13247, 0.06509327318403745899 ) ;
#2801=VERTEX_POINT ( 'NONE', #118883 ) ;
#2802=ORIENTED_EDGE ( 'NONE', *, *, #13755, .F. ) ;
#2803=EDGE_LOOP ( 'NONE', ( #104737, #104794, #73009, #19513 ) ) ;
#2804=AXIS2_PLACEMENT_3D ( 'NONE', #112969, #15396, #3663 ) ;
#2805=CARTESIAN_POINT ( 'NONE',  ( 11.04999999999990656, 2.500000000000000000, 2.511473670974873507 ) ) ;
#2806=CARTESIAN_POINT ( 'NONE',  ( -4.350000000000023626, 2.500000000000000000, 6.741600689897071952 ) ) ;
#2807=EDGE_CURVE ( 'NONE', #124598, #74378, #113134, .T. ) ;
#2808=VECTOR ( 'NONE', #86278, 1000.000000000000000 ) ;
#2809=DIRECTION ( 'NONE',  ( -0.000000000000000000, -1.000000000000000000, -0.000000000000000000 ) ) ;
#2810=LINE ( 'NONE', #21823, #28219 ) ;
#2811=CIRCLE ( 'NONE', #75956, 0.06509327318403745899 ) ;
#2812=CIRCLE ( 'NONE', #40488, 0.09999999999999982514 ) ;
#2813=DIRECTION ( 'NONE',  ( -0.000000000000000000, -1.000000000000000000, -0.000000000000000000 ) ) ;
#2814=DIRECTION ( 'NONE',  ( 0.000000000000000000, 0.000000000000000000, -1.000000000000000000 ) ) ;
#2815=CIRCLE ( 'NONE', #78030, 0.06509327318403745899 ) ;
#2816=ORIENTED_EDGE ( 'NONE', *, *, #26281, .F. ) ;
#2817=DIRECTION ( 'NONE',  ( -0.000000000000000000, 1.000000000000000000, -0.000000000000000000 ) ) ;
#2818=CIRCLE ( 'NONE', #57097, 0.06509327318403745899 ) ;
#2819=EDGE_LOOP ( 'NONE', ( #1407, #66731, #34191, #113258 ) ) ;
#2820=CARTESIAN_POINT ( 'NONE',  ( -7.500000000000001776, -1.500000000000000000, 1.734723475976807094E-15 ) ) ;
#2821=AXIS2_PLACEMENT_3D ( 'NONE', #94067, #35792, #84886 ) ;
#2822=VERTEX_POINT ( 'NONE', #52084 ) ;
#2823=AXIS2_PLACEMENT_3D ( 'NONE', #115984, #76708, #87799 ) ;
#2824=DIRECTION ( 'NONE',  ( 0.000000000000000000, 0.000000000000000000, 1.000000000000000000 ) ) ;
#2825=ADVANCED_FACE ( 'NONE', ( #39060 ), #79782, .T. ) ;
#2826=VERTEX_POINT ( 'NONE', #78973 ) ;
#2827=CIRCLE ( 'NONE', #54753, 0.06509327318403745899 ) ;
#2829=DIRECTION ( 'NONE',  ( -4.274815082592931898E-19, -0.9999939076577903929, -0.003490651415223739937 ) ) ;
#2830=VERTEX_POINT ( 'NONE', #71712 ) ;
#2831=ORIENTED_EDGE ( 'NONE', *, *, #96438, .T. ) ;
#2832=CARTESIAN_POINT ( 'NONE',  ( 5.449999999999937117, 12.50000000000000000, -6.495190528383302464 ) ) ;
#2833=CARTESIAN_POINT ( 'NONE',  ( -12.29999999999999716, 2.500000000000000000, -3.983716857408423628 ) ) ;
#2835=CARTESIAN_POINT ( 'NONE',  ( -10.60000000000000142, 2.500000000000000000, 4.676537180435972552 ) ) ;
#2836=DIRECTION ( 'NONE',  ( 0.000000000000000000, 0.000000000000000000, -1.000000000000000000 ) ) ;
#2837=AXIS2_PLACEMENT_3D ( 'NONE', #12525, #32840, #52452 ) ;
#2838=DIRECTION ( 'NONE',  ( -0.000000000000000000, -1.000000000000000000, -0.000000000000000000 ) ) ;
#2839=VERTEX_POINT ( 'NONE', #80255 ) ;
#2840=DIRECTION ( 'NONE',  ( 0.000000000000000000, 0.000000000000000000, -1.000000000000000000 ) ) ;
#2841=AXIS2_PLACEMENT_3D ( 'NONE', #52286, #101390, #42477 ) ;
#2842=ORIENTED_EDGE ( 'NONE', *, *, #51787, .F. ) ;
#2843=DIRECTION ( 'NONE',  ( 0.000000000000000000, 1.000000000000000000, 0.000000000000000000 ) ) ;
#2844=CARTESIAN_POINT ( 'NONE',  ( 8.949999999999919353, 2.500000000000000000, 2.511473670974873507 ) ) ;
#2845=CONICAL_SURFACE ( 'NONE', #65529, 0.1000000000000002554, 0.003490658503988666988 ) ;
#2846=EDGE_CURVE ( 'NONE', #103729, #127557, #17039, .T. ) ;
#2848=CARTESIAN_POINT ( 'NONE',  ( 2.949999999999946887, 2.500000000000000000, -6.595190528383302109 ) ) ;
#2849=CARTESIAN_POINT ( 'NONE',  ( 5.399999999999934630, 2.500000000000000000, -0.6928203230275542523 ) ) ;
#2850=CARTESIAN_POINT ( 'NONE',  ( -9.150000000000005684, 2.500000000000000000, 6.395190528383296602 ) ) ;
#2851=AXIS2_PLACEMENT_3D ( 'NONE', #28162, #100745, #9809 ) ;
#2852=FACE_OUTER_BOUND ( 'NONE', #47678, .T. ) ;
#2853=VECTOR ( 'NONE', #71076, 1000.000000000000000 ) ;
#2854=VERTEX_POINT ( 'NONE', #111645 ) ;
#2855=CIRCLE ( 'NONE', #107312, 0.09999999999999982514 ) ;
#2856=EDGE_CURVE ( 'NONE', #125867, #129536, #86020, .T. ) ;
#2857=CIRCLE ( 'NONE', #36334, 0.1000000000000002554 ) ;
#2858=DIRECTION ( 'NONE',  ( 0.000000000000000000, 0.000000000000000000, 1.000000000000000000 ) ) ;
#2859=LINE ( 'NONE', #31677, #69334 ) ;
#2860=DIRECTION ( 'NONE',  ( 0.000000000000000000, 0.000000000000000000, 1.000000000000000000 ) ) ;
#2861=ORIENTED_EDGE ( 'NONE', *, *, #8471, .F. ) ;
#2862=EDGE_CURVE ( 'NONE', #32372, #94541, #109009, .T. ) ;
#2863=EDGE_CURVE ( 'NONE', #59036, #43078, #11504, .T. ) ;
#2864=EDGE_CURVE ( 'NONE', #64833, #125995, #67522, .T. ) ;
#2866=ADVANCED_FACE ( 'NONE', ( #99894 ), #117406, .T. ) ;
#2867=CARTESIAN_POINT ( 'NONE',  ( -0.8000000000000381251, 2.500000000000000000, 4.330127018922196314 ) ) ;
#2869=CONICAL_SURFACE ( 'NONE', #13315, 0.1000000000000000472, 0.003490658503988666988 ) ;
#2870=VECTOR ( 'NONE', #31644, 1000.000000000000000 ) ;
#2871=EDGE_LOOP ( 'NONE', ( #39620, #38671 ) ) ;
#2872=AXIS2_PLACEMENT_3D ( 'NONE', #48187, #76367, #78954 ) ;
#2873=CARTESIAN_POINT ( 'NONE',  ( -5.650000000000019895, 12.50000000000000000, 1.753560074763284016 ) ) ;
#2874=EDGE_CURVE ( 'NONE', #102170, #108113, #49514, .T. ) ;
#2875=EDGE_CURVE ( 'NONE', #86508, #71451, #27527, .T. ) ;
#2876=VECTOR ( 'NONE', #127363, 1000.000000000000000 ) ;
#2877=ORIENTED_EDGE ( 'NONE', *, *, #55480, .T. ) ;
#2878=CARTESIAN_POINT ( 'NONE',  ( 19.51231976789051004, -0.5900868802302308147, -4.348342248683373157 ) ) ;
#2880=ADVANCED_FACE ( 'NONE', ( #20050 ), #31797, .T. ) ;
#2881=DIRECTION ( 'NONE',  ( 0.000000000000000000, 1.000000000000000000, 0.000000000000000000 ) ) ;
#2882=AXIS2_PLACEMENT_3D ( 'NONE', #45406, #23829, #104315 ) ;
#2883=EDGE_LOOP ( 'NONE', ( #50197, #22597, #38292, #93513 ) ) ;
#2884=EDGE_CURVE ( 'NONE', #117215, #36888, #46324, .T. ) ;
#2885=CARTESIAN_POINT ( 'NONE',  ( 4.599999999999940137, 12.50000000000000000, -4.330127018922201643 ) ) ;
#2886=ADVANCED_FACE ( 'NONE', ( #61911 ), #12133, .T. ) ;
#2887=DIRECTION ( 'NONE',  ( 0.000000000000000000, -0.000000000000000000, 1.000000000000000000 ) ) ;
#2888=EDGE_CURVE ( 'NONE', #110892, #7910, #345, .T. ) ;
#2889=EDGE_LOOP ( 'NONE', ( #97506, #30568, #102218, #60719 ) ) ;
#2890=VERTEX_POINT ( 'NONE', #101823 ) ;
#2891=ORIENTED_EDGE ( 'NONE', *, *, #36717, .F. ) ;
#2892=DIRECTION ( 'NONE',  ( 0.000000000000000000, 1.000000000000000000, 0.000000000000000000 ) ) ;
#2893=CARTESIAN_POINT ( 'NONE',  ( 0.1999999999999562961, 2.500000000000000000, 4.776537180435972196 ) ) ;
#2894=AXIS2_PLACEMENT_3D ( 'NONE', #39859, #537, #69942 ) ;
#2895=DIRECTION ( 'NONE',  ( 0.000000000000000000, 0.000000000000000000, 1.000000000000000000 ) ) ;
#2896=AXIS2_PLACEMENT_3D ( 'NONE', #37229, #48989, #86953 ) ;
#2897=FACE_BOUND ( 'NONE', #83659, .T. ) ;
#2898=ORIENTED_EDGE ( 'NONE', *, *, #88134, .F. ) ;
#2899=DIRECTION ( 'NONE',  ( -0.000000000000000000, 1.000000000000000000, -0.000000000000000000 ) ) ;
#2900=DIRECTION ( 'NONE',  ( 0.000000000000000000, 1.000000000000000000, 0.000000000000000000 ) ) ;
#2901=ORIENTED_EDGE ( 'NONE', *, *, #54875, .F. ) ;
#2902=CARTESIAN_POINT ( 'NONE',  ( -13.74999999999995381, 2.500000000000000000, -2.165063509461099489 ) ) ;
#2903=CONICAL_SURFACE ( 'NONE', #96982, 0.09999999999999982514, 0.003490658503988666988 ) ;
#2904=DIRECTION ( 'NONE',  ( 0.000000000000000000, 0.000000000000000000, -1.000000000000000000 ) ) ;
#2905=CIRCLE ( 'NONE', #101097, 0.09999999999999999167 ) ;
#2906=CONICAL_SURFACE ( 'NONE', #21791, 0.09999999999999982514, 0.003490658503988666988 ) ;
#2907=AXIS2_PLACEMENT_3D ( 'NONE', #125304, #95204, #44823 ) ;
#2908=FACE_OUTER_BOUND ( 'NONE', #54465, .T. ) ;
#2909=CONICAL_SURFACE ( 'NONE', #65594, 0.1000000000000002554, 0.003490658503988666988 ) ;
#2910=DIRECTION ( 'NONE',  ( 0.000000000000000000, 1.000000000000000000, 0.000000000000000000 ) ) ;
#2911=DIRECTION ( 'NONE',  ( 0.000000000000000000, 0.000000000000000000, -1.000000000000000000 ) ) ;
#2912=CARTESIAN_POINT ( 'NONE',  ( -13.34999999999999076, 12.50000000000000000, 2.230156782645138946 ) ) ;
#2913=DIRECTION ( 'NONE',  ( 0.000000000000000000, 1.000000000000000000, 0.000000000000000000 ) ) ;
#2914=CIRCLE ( 'NONE', #61508, 0.09999999999999999167 ) ;
#2915=CIRCLE ( 'NONE', #92808, 0.1000000000000002554 ) ;
#2916=AXIS2_PLACEMENT_3D ( 'NONE', #53932, #34307, #93855 ) ;
#2917=ORIENTED_EDGE ( 'NONE', *, *, #98468, .F. ) ;
#2918=ORIENTED_EDGE ( 'NONE', *, *, #82838, .T. ) ;
#2919=EDGE_LOOP ( 'NONE', ( #31296, #7476, #64231, #72085 ) ) ;
#2920=ORIENTED_EDGE ( 'NONE', *, *, #18343, .F. ) ;
#2921=DIRECTION ( 'NONE',  ( 0.000000000000000000, 1.000000000000000000, 0.000000000000000000 ) ) ;
#2923=CIRCLE ( 'NONE', #107370, 0.06509327318403745899 ) ;
#2924=DIRECTION ( 'NONE',  ( 0.000000000000000000, 0.000000000000000000, -1.000000000000000000 ) ) ;
#2925=EDGE_LOOP ( 'NONE', ( #125324, #46202, #20469, #66864 ) ) ;
#2926=FACE_BOUND ( 'NONE', #55172, .T. ) ;
#2927=CARTESIAN_POINT ( 'NONE',  ( -3.350000000000031619, 2.500000000000000000, -7.188010851410854052 ) ) ;
#2928=DIRECTION ( 'NONE',  ( -0.000000000000000000, -1.000000000000000000, -0.000000000000000000 ) ) ;
#2929=EDGE_CURVE ( 'NONE', #124072, #104109, #67218, .T. ) ;
#2930=DIRECTION ( 'NONE',  ( -0.000000000000000000, -1.000000000000000000, -0.000000000000000000 ) ) ;
#2931=FACE_OUTER_BOUND ( 'NONE', #11110, .T. ) ;
#2932=EDGE_CURVE ( 'NONE', #74283, #269, #33102, .T. ) ;
#2933=LINE ( 'NONE', #23195, #109876 ) ;
#2934=CARTESIAN_POINT ( 'NONE',  ( -14.14999999999998614, 12.50000000000000000, -2.165063509461099489 ) ) ;
#2935=CARTESIAN_POINT ( 'NONE',  ( 1.649999999999949729, 2.500000000000000000, 5.702370205355745014 ) ) ;
#2936=CARTESIAN_POINT ( 'NONE',  ( -4.400000000000028777, 2.500000000000000000, -4.576537180435978236 ) ) ;
#2937=CARTESIAN_POINT ( 'NONE',  ( 8.949999999999919353, 2.500000000000000000, 2.511473670974873507 ) ) ;
#2938=VECTOR ( 'NONE', #127645, 1000.000000000000000 ) ;
#2939=EDGE_CURVE ( 'NONE', #4198, #42202, #113221, .T. ) ;
#2940=ORIENTED_EDGE ( 'NONE', *, *, #2076, .F. ) ;
#2941=ORIENTED_EDGE ( 'NONE', *, *, #3346, .F. ) ;
#2942=ORIENTED_EDGE ( 'NONE', *, *, #79157, .T. ) ;
#2943=ORIENTED_EDGE ( 'NONE', *, *, #58252, .T. ) ;
#2944=EDGE_LOOP ( 'NONE', ( #46310, #51820, #113043, #48664 ) ) ;
#2945=VERTEX_POINT ( 'NONE', #4241 ) ;
#2946=CARTESIAN_POINT ( 'NONE',  ( -14.14999999999998614, 2.500000000000000000, -2.857883832488651521 ) ) ;
#2947=ORIENTED_EDGE ( 'NONE', *, *, #29388, .F. ) ;
#2948=VERTEX_POINT ( 'NONE', #14058 ) ;
#2949=CONICAL_SURFACE ( 'NONE', #76098, 0.1000000000000000472, 0.003490658503988666988 ) ;
#2950=DIRECTION ( 'NONE',  ( 0.000000000000000000, 1.000000000000000000, 0.000000000000000000 ) ) ;
#2951=LINE ( 'NONE', #102438, #12345 ) ;
#2952=CARTESIAN_POINT ( 'NONE',  ( -2.100000000000033396, 2.500000000000000000, 0.5928203230275495006 ) ) ;
#2953=AXIS2_PLACEMENT_3D ( 'NONE', #13504, #80976, #122195 ) ;
#2954=VERTEX_POINT ( 'NONE', #32469 ) ;
#2956=AXIS2_PLACEMENT_3D ( 'NONE', #50760, #111609, #72348 ) ;
#2957=EDGE_LOOP ( 'NONE', ( #63891, #4320, #122732, #39382 ) ) ;
#2958=AXIS2_PLACEMENT_3D ( 'NONE', #114890, #114256, #34430 ) ;
#2959=VERTEX_POINT ( 'NONE', #52714 ) ;
#2960=LINE ( 'NONE', #1015, #126233 ) ;
#2961=DIRECTION ( 'NONE',  ( -0.000000000000000000, -1.000000000000000000, -0.000000000000000000 ) ) ;
#2962=ORIENTED_EDGE ( 'NONE', *, *, #66844, .F. ) ;
#2963=VERTEX_POINT ( 'NONE', #14701 ) ;
#2964=PLANE ( 'NONE',  #84041 ) ;
#2965=DIRECTION ( 'NONE',  ( 0.000000000000000000, 0.000000000000000000, 1.000000000000000000 ) ) ;
#2966=AXIS2_PLACEMENT_3D ( 'NONE', #23650, #100281, #86426 ) ;
#2967=CARTESIAN_POINT ( 'NONE',  ( 6.699999999999928235, 2.500000000000000000, -2.276824562219559311E-15 ) ) ;
#2968=CIRCLE ( 'NONE', #76120, 0.09999999999999982514 ) ;
#2969=VECTOR ( 'NONE', #49915, 1000.000000000000000 ) ;
#2970=DIRECTION ( 'NONE',  ( 0.000000000000000000, -0.9999939076577903929, 0.003490651415223739937 ) ) ;
#2971=DIRECTION ( 'NONE',  ( 0.000000000000000000, 1.000000000000000000, 0.000000000000000000 ) ) ;
#2972=VECTOR ( 'NONE', #65029, 1000.000000000000000 ) ;
#2973=ORIENTED_EDGE ( 'NONE', *, *, #92624, .T. ) ;
#2974=AXIS2_PLACEMENT_3D ( 'NONE', #52789, #122189, #92724 ) ;
#2975=DIRECTION ( 'NONE',  ( -4.274815082592931898E-19, -0.9999939076577903929, -0.003490651415223739937 ) ) ;
#2976=ORIENTED_EDGE ( 'NONE', *, *, #26758, .T. ) ;
#2978=ORIENTED_EDGE ( 'NONE', *, *, #44260, .F. ) ;
#2979=FACE_OUTER_BOUND ( 'NONE', #124618, .T. ) ;
#2980=DIRECTION ( 'NONE',  ( 0.000000000000000000, 0.000000000000000000, 1.000000000000000000 ) ) ;
#2981=EDGE_CURVE ( 'NONE', #62375, #7926, #50525, .T. ) ;
#2983=EDGE_CURVE ( 'NONE', #58412, #8031, #122747, .T. ) ;
#2984=DIRECTION ( 'NONE',  ( 0.000000000000000000, -0.9999939076577903929, 0.003490651415223739937 ) ) ;
#2985=VERTEX_POINT ( 'NONE', #35035 ) ;
#2986=CARTESIAN_POINT ( 'NONE',  ( -5.650000000000023448, 12.50000000000000000, -2.511473670974877948 ) ) ;
#2987=AXIS2_PLACEMENT_3D ( 'NONE', #52892, #111820, #73806 ) ;
#2988=CARTESIAN_POINT ( 'NONE',  ( -6.450000000000014388, 2.500000000000000000, 1.818653347947321475 ) ) ;
#2989=VERTEX_POINT ( 'NONE', #25181 ) ;
#2990=VERTEX_POINT ( 'NONE', #83484 ) ;
#2991=AXIS2_PLACEMENT_3D ( 'NONE', #119516, #88780, #128735 ) ;
#2992=ADVANCED_FACE ( 'NONE', ( #24545 ), #69299, .T. ) ;
#2993=ORIENTED_EDGE ( 'NONE', *, *, #72344, .F. ) ;
#2994=CARTESIAN_POINT ( 'NONE',  ( 17.50000000000000000, -2.750000000000000444, 2.864912725862981624 ) ) ;
#2995=CARTESIAN_POINT ( 'NONE',  ( -11.84999999999999609, 12.50000000000000000, 2.511473670974873507 ) ) ;
#2997=DIRECTION ( 'NONE',  ( -4.274815082592931898E-19, -0.9999939076577903929, -0.003490651415223739937 ) ) ;
#2998=DIRECTION ( 'NONE',  ( 0.000000000000000000, 0.000000000000000000, -1.000000000000000000 ) ) ;
#2999=AXIS2_PLACEMENT_3D ( 'NONE', #115365, #67568, #8641 ) ;
#3000=CIRCLE ( 'NONE', #76154, 0.1000000000000000472 ) ;
#3001=CARTESIAN_POINT ( 'NONE',  ( 5.599999999999931255, 12.50000000000000000, 4.611443907251934426 ) ) ;
#3002=CIRCLE ( 'NONE', #49075, 0.06509327318403745899 ) ;
#3003=DIRECTION ( 'NONE',  ( 0.000000000000000000, 0.000000000000000000, -1.000000000000000000 ) ) ;
#3004=VECTOR ( 'NONE', #101494, 1000.000000000000000 ) ;
#3005=CIRCLE ( 'NONE', #59164, 0.09999999999999999167 ) ;
#3006=VECTOR ( 'NONE', #128243, 1000.000000000000000 ) ;
#3007=FACE_OUTER_BOUND ( 'NONE', #64248, .T. ) ;
#3008=AXIS2_PLACEMENT_3D ( 'NONE', #89189, #19810, #28993 ) ;
#3009=EDGE_LOOP ( 'NONE', ( #20545, #20901, #29975, #29772 ) ) ;
#3010=CARTESIAN_POINT ( 'NONE',  ( 10.64999999999991331, 12.50000000000000000, 6.148780366869520897 ) ) ;
#3011=AXIS2_PLACEMENT_3D ( 'NONE', #16316, #66718, #57568 ) ;
#3012=FACE_OUTER_BOUND ( 'NONE', #114721, .T. ) ;
#3013=DIRECTION ( 'NONE',  ( 0.000000000000000000, 1.000000000000000000, 0.000000000000000000 ) ) ;
#3014=CARTESIAN_POINT ( 'NONE',  ( -12.89999999999999147, 2.500000000000000000, -4.430127018922199511 ) ) ;
#3015=ORIENTED_EDGE ( 'NONE', *, *, #25209, .T. ) ;
#3016=DIRECTION ( 'NONE',  ( 0.000000000000000000, 0.000000000000000000, -1.000000000000000000 ) ) ;
#3017=EDGE_CURVE ( 'NONE', #116336, #76857, #102465, .T. ) ;
#3018=DIRECTION ( 'NONE',  ( 0.000000000000000000, 1.000000000000000000, 0.000000000000000000 ) ) ;
#3019=CARTESIAN_POINT ( 'NONE',  ( -4.550000000000022915, 2.500000000000000000, 2.065063509461097624 ) ) ;
#3020=ORIENTED_EDGE ( 'NONE', *, *, #25234, .F. ) ;
#3021=EDGE_CURVE ( 'NONE', #64709, #48204, #114844, .T. ) ;
#3022=ADVANCED_FACE ( 'NONE', ( #65094 ), #7579, .T. ) ;
#3023=EDGE_CURVE ( 'NONE', #116228, #101562, #107943, .T. ) ;
#3025=AXIS2_PLACEMENT_3D ( 'NONE', #13275, #129391, #93151 ) ;
#3026=ORIENTED_EDGE ( 'NONE', *, *, #45395, .T. ) ;
#3028=ORIENTED_EDGE ( 'NONE', *, *, #25160, .T. ) ;
#3029=ORIENTED_EDGE ( 'NONE', *, *, #63770, .F. ) ;
#3030=DIRECTION ( 'NONE',  ( 0.000000000000000000, 0.000000000000000000, -1.000000000000000000 ) ) ;
#3031=ADVANCED_FACE ( 'NONE', ( #74300 ), #24316, .T. ) ;
#3032=EDGE_CURVE ( 'NONE', #54523, #77368, #112292, .T. ) ;
#3033=FACE_OUTER_BOUND ( 'NONE', #126812, .T. ) ;
#3034=CARTESIAN_POINT ( 'NONE',  ( 11.04999999999991189, 2.500000000000000000, -2.511473670974877948 ) ) ;
#3035=CONICAL_SURFACE ( 'NONE', #76199, 0.09999999999999982514, 0.003490658503988666988 ) ;
#3036=DIRECTION ( 'NONE',  ( -4.274815082592931898E-19, -0.9999939076577903929, -0.003490651415223739937 ) ) ;
#3037=AXIS2_PLACEMENT_3D ( 'NONE', #117006, #94815, #95461 ) ;
#3038=ORIENTED_EDGE ( 'NONE', *, *, #37626, .F. ) ;
#3039=ADVANCED_FACE ( 'NONE', ( #2979 ), #120464, .T. ) ;
#3040=DIRECTION ( 'NONE',  ( -0.000000000000000000, -1.000000000000000000, -0.000000000000000000 ) ) ;
#3041=DIRECTION ( 'NONE',  ( 0.000000000000000000, 0.000000000000000000, 1.000000000000000000 ) ) ;
#3042=VERTEX_POINT ( 'NONE', #44844 ) ;
#3043=CARTESIAN_POINT ( 'NONE',  ( -4.400000000000025224, 2.500000000000000000, -0.3464101615137783474 ) ) ;
#3044=EDGE_CURVE ( 'NONE', #6762, #4367, #57777, .T. ) ;
#3045=PLANE ( 'NONE',  #46671 ) ;
#3046=EDGE_CURVE ( 'NONE', #52919, #15089, #74493, .T. ) ;
#3047=EDGE_LOOP ( 'NONE', ( #37865, #56529 ) ) ;
#3048=CIRCLE ( 'NONE', #894, 0.1000000000000002554 ) ;
#3049=EDGE_LOOP ( 'NONE', ( #103305, #32878, #103032, #76036 ) ) ;
#3050=AXIS2_PLACEMENT_3D ( 'NONE', #94328, #94996, #75989 ) ;
#3051=VERTEX_POINT ( 'NONE', #82843 ) ;
#3052=ORIENTED_EDGE ( 'NONE', *, *, #92624, .F. ) ;
#3053=FACE_OUTER_BOUND ( 'NONE', #37505, .T. ) ;
#3054=CARTESIAN_POINT ( 'NONE',  ( 16.04744068708516025, 2.499999999999872546, 6.586254740842515609 ) ) ;
#3055=CARTESIAN_POINT ( 'NONE',  ( -11.05000000000000071, 12.50000000000000000, -2.576566944158911188 ) ) ;
#3056=FACE_BOUND ( 'NONE', #124023, .T. ) ;
#3057=ORIENTED_EDGE ( 'NONE', *, *, #18254, .F. ) ;
#3059=CARTESIAN_POINT ( 'NONE',  ( -2.300000000000032685, 2.500000000000000000, -0.3464101615137783474 ) ) ;
#3060=CARTESIAN_POINT ( 'NONE',  ( -2.950000000000030376, 12.50000000000000000, 6.430097255199259010 ) ) ;
#3061=AXIS2_PLACEMENT_3D ( 'NONE', #37978, #34461, #10451 ) ;
#3062=AXIS2_PLACEMENT_3D ( 'NONE', #119924, #70185, #20434 ) ;
#3063=DIRECTION ( 'NONE',  ( 0.000000000000000000, -0.9999939076577903929, 0.003490651415223739937 ) ) ;
#3064=DIRECTION ( 'NONE',  ( 0.000000000000000000, -0.9999939076577903929, 0.003490651415223739937 ) ) ;
#3065=AXIS2_PLACEMENT_3D ( 'NONE', #91139, #1457, #12561 ) ;
#3066=FACE_OUTER_BOUND ( 'NONE', #14518, .T. ) ;
#3068=DIRECTION ( 'NONE',  ( 0.000000000000000000, 1.000000000000000000, 0.000000000000000000 ) ) ;
#3069=ORIENTED_EDGE ( 'NONE', *, *, #64210, .F. ) ;
#3070=VERTEX_POINT ( 'NONE', #73004 ) ;
#3071=VERTEX_POINT ( 'NONE', #94564 ) ;
#3072=VERTEX_POINT ( 'NONE', #68334 ) ;
#3073=ORIENTED_EDGE ( 'NONE', *, *, #99203, .F. ) ;
#3074=DIRECTION ( 'NONE',  ( 0.000000000000000000, 1.000000000000000000, 0.000000000000000000 ) ) ;
#3075=DIRECTION ( 'NONE',  ( 0.000000000000000000, 0.000000000000000000, 1.000000000000000000 ) ) ;
#3076=VERTEX_POINT ( 'NONE', #46776 ) ;
#3077=FACE_BOUND ( 'NONE', #112096, .T. ) ;
#3078=FACE_OUTER_BOUND ( 'NONE', #69946, .T. ) ;
#3079=EDGE_CURVE ( 'NONE', #29857, #85157, #97479, .T. ) ;
#3080=AXIS2_PLACEMENT_3D ( 'NONE', #29399, #68662, #129548 ) ;
#3081=AXIS2_PLACEMENT_3D ( 'NONE', #37127, #124854, #65920 ) ;
#3082=ADVANCED_FACE ( 'NONE', ( #125325 ), #70299, .T. ) ;
#3083=AXIS2_PLACEMENT_3D ( 'NONE', #36324, #36955, #34392 ) ;
#3084=VERTEX_POINT ( 'NONE', #67025 ) ;
#3085=AXIS2_PLACEMENT_3D ( 'NONE', #32267, #20012, #59958 ) ;
#3086=CARTESIAN_POINT ( 'NONE',  ( -0.8500000000000382805, 2.500000000000000000, -5.802370205355749988 ) ) ;
#3087=CARTESIAN_POINT ( 'NONE',  ( 14.14999999999989200, 2.500000000000000000, -2.165063509461101710 ) ) ;
#3088=CARTESIAN_POINT ( 'NONE',  ( 3.549999999999944755, 2.500000000000000000, -2.411473670974877859 ) ) ;
#3089=ORIENTED_EDGE ( 'NONE', *, *, #82819, .T. ) ;
#3090=CARTESIAN_POINT ( 'NONE',  ( 9.349999999999916156, 12.50000000000000000, -2.576566944158915184 ) ) ;
#3091=CONICAL_SURFACE ( 'NONE', #126331, 0.09999999999999982514, 0.003490658503988666988 ) ;
#3092=ORIENTED_EDGE ( 'NONE', *, *, #13804, .T. ) ;
#3093=CONICAL_SURFACE ( 'NONE', #99240, 0.09999999999999982514, 0.003490658503988666988 ) ;
#3094=ORIENTED_EDGE ( 'NONE', *, *, #84045, .F. ) ;
#3095=ORIENTED_EDGE ( 'NONE', *, *, #111499, .F. ) ;
#3096=DIRECTION ( 'NONE',  ( 0.000000000000000000, 1.000000000000000000, 0.000000000000000000 ) ) ;
#3097=DIRECTION ( 'NONE',  ( -0.000000000000000000, -1.000000000000000000, -0.000000000000000000 ) ) ;
#3098=DIRECTION ( 'NONE',  ( -0.000000000000000000, -1.000000000000000000, -0.000000000000000000 ) ) ;
#3099=EDGE_LOOP ( 'NONE', ( #37012, #43985 ) ) ;
#3100=LINE ( 'NONE', #123496, #99753 ) ;
#3101=CIRCLE ( 'NONE', #63737, 0.06509327318403743123 ) ;
#3102=VECTOR ( 'NONE', #47038, 1000.000000000000000 ) ;
#3103=CARTESIAN_POINT ( 'NONE',  ( 11.89999999999990798, 2.500000000000000000, 3.983716857408420964 ) ) ;
#3104=FACE_OUTER_BOUND ( 'NONE', #129495, .T. ) ;
#3106=CONICAL_SURFACE ( 'NONE', #76263, 0.1000000000000002554, 0.003490658503988666988 ) ;
#3107=VERTEX_POINT ( 'NONE', #57226 ) ;
#3108=DIRECTION ( 'NONE',  ( 0.000000000000000000, 1.000000000000000000, 0.000000000000000000 ) ) ;
#3109=EDGE_LOOP ( 'NONE', ( #35902, #44593, #14054, #105016 ) ) ;
#3110=CARTESIAN_POINT ( 'NONE',  ( 6.249999999999965361, 12.50000000000000000, 2.165063509461097713 ) ) ;
#3111=EDGE_LOOP ( 'NONE', ( #75458, #9768 ) ) ;
#3112=VERTEX_POINT ( 'NONE', #77510 ) ;
#3113=CARTESIAN_POINT ( 'NONE',  ( 14.14999999999989733, 2.500000000000000000, 2.757883832488649656 ) ) ;
#3114=DIRECTION ( 'NONE',  ( 0.000000000000000000, 0.000000000000000000, 1.000000000000000000 ) ) ;
#3115=DIRECTION ( 'NONE',  ( 0.000000000000000000, -0.9999939076577903929, 0.003490651415223739937 ) ) ;
#3116=DIRECTION ( 'NONE',  ( -0.000000000000000000, 1.000000000000000000, -0.000000000000000000 ) ) ;
#3117=DIRECTION ( 'NONE',  ( 0.000000000000000000, 0.000000000000000000, 1.000000000000000000 ) ) ;
#3118=CONICAL_SURFACE ( 'NONE', #80578, 0.09999999999999982514, 0.003490658503988666988 ) ;
#3119=EDGE_LOOP ( 'NONE', ( #89447, #27038 ) ) ;
#3120=VERTEX_POINT ( 'NONE', #95229 ) ;
#3121=EDGE_CURVE ( 'NONE', #76595, #38808, #22287, .T. ) ;
#3122=CARTESIAN_POINT ( 'NONE',  ( 12.69999999999990337, 2.500000000000000000, -4.776537180435978414 ) ) ;
#3124=FACE_OUTER_BOUND ( 'NONE', #45226, .T. ) ;
#3125=VERTEX_POINT ( 'NONE', #38248 ) ;
#3126=ORIENTED_EDGE ( 'NONE', *, *, #54598, .T. ) ;
#3127=CARTESIAN_POINT ( 'NONE',  ( 10.84999999999990905, 2.500000000000000000, -5.702370205355749455 ) ) ;
#3128=AXIS2_PLACEMENT_3D ( 'NONE', #80850, #53330, #120767 ) ;
#3129=ORIENTED_EDGE ( 'NONE', *, *, #112470, .F. ) ;
#3130=CARTESIAN_POINT ( 'NONE',  ( 8.749999999999923617, 12.50000000000000000, 1.472243186433545459 ) ) ;
#3131=ADVANCED_FACE ( 'NONE', ( #127905 ), #85398, .T. ) ;
#3132=CARTESIAN_POINT ( 'NONE',  ( -6.650000000000018119, 12.50000000000000000, -2.165063509461101710 ) ) ;
#3133=CONICAL_SURFACE ( 'NONE', #53309, 0.1000000000000002554, 0.003490658503988666988 ) ;
#3134=CARTESIAN_POINT ( 'NONE',  ( 2.899999999999944844, 2.500000000000000000, 3.737306695894644371 ) ) ;
#3135=VERTEX_POINT ( 'NONE', #75569 ) ;
#3136=PLANE ( 'NONE',  #92070 ) ;
#3137=DIRECTION ( 'NONE',  ( 0.000000000000000000, 0.000000000000000000, -1.000000000000000000 ) ) ;
#3138=CARTESIAN_POINT ( 'NONE',  ( 14.54999999999989591, 2.500000000000000000, 2.165063509461097713 ) ) ;
#3139=CARTESIAN_POINT ( 'NONE',  ( 1.449999999999949551, 2.500000000000000000, 6.941600689897073018 ) ) ;
#3140=ADVANCED_FACE ( 'NONE', ( #76235 ), #28528, .T. ) ;
#3142=CARTESIAN_POINT ( 'NONE',  ( 5.799999999999931433, 2.500000000000000000, 4.330127018922196314 ) ) ;
#3143=EDGE_LOOP ( 'NONE', ( #79118, #76165, #78870, #53190 ) ) ;
#3144=AXIS2_PLACEMENT_3D ( 'NONE', #3514, #43453, #64357 ) ;
#3145=DIRECTION ( 'NONE',  ( 0.000000000000000000, 0.000000000000000000, -1.000000000000000000 ) ) ;
#3146=CARTESIAN_POINT ( 'NONE',  ( 81.97643238289522571, -3.858501988011899364, 6.173828414998187242 ) ) ;
#3147=AXIS2_PLACEMENT_3D ( 'NONE', #40616, #32719, #100768 ) ;
#3148=EDGE_LOOP ( 'NONE', ( #36468, #56392, #8981, #100650 ) ) ;
#3150=EDGE_CURVE ( 'NONE', #46254, #96832, #45252, .T. ) ;
#3152=DIRECTION ( 'NONE',  ( 0.000000000000000000, -0.000000000000000000, 1.000000000000000000 ) ) ;
#3153=DIRECTION ( 'NONE',  ( 0.000000000000000000, 0.000000000000000000, 1.000000000000000000 ) ) ;
#3154=PLANE ( 'NONE',  #84551 ) ;
#3155=CARTESIAN_POINT ( 'NONE',  ( -0.8000000000000315747, 12.50000000000000000, 0.000000000000000000 ) ) ;
#3156=VECTOR ( 'NONE', #88026, 1000.000000000000000 ) ;
#3157=FACE_OUTER_BOUND ( 'NONE', #125977, .T. ) ;
#3158=AXIS2_PLACEMENT_3D ( 'NONE', #12720, #52033, #51401 ) ;
#3159=CARTESIAN_POINT ( 'NONE',  ( -0.2000000000000347888, 12.50000000000000000, 0.4115034346978132529 ) ) ;
#3160=DIRECTION ( 'NONE',  ( -0.000000000000000000, 1.000000000000000000, -0.000000000000000000 ) ) ;
#3161=DIRECTION ( 'NONE',  ( 0.000000000000000000, 0.000000000000000000, 1.000000000000000000 ) ) ;
#3163=ORIENTED_EDGE ( 'NONE', *, *, #14410, .T. ) ;
#3164=VERTEX_POINT ( 'NONE', #27129 ) ;
#3165=ORIENTED_EDGE ( 'NONE', *, *, #101283, .T. ) ;
#3166=ORIENTED_EDGE ( 'NONE', *, *, #62858, .T. ) ;
#3167=AXIS2_PLACEMENT_3D ( 'NONE', #106632, #17599, #57544 ) ;
#3168=DIRECTION ( 'NONE',  ( 0.000000000000000000, 1.000000000000000000, 0.000000000000000000 ) ) ;
#3169=DIRECTION ( 'NONE',  ( 0.000000000000000000, 0.000000000000000000, 1.000000000000000000 ) ) ;
#3170=ORIENTED_EDGE ( 'NONE', *, *, #30964, .F. ) ;
#3171=DIRECTION ( 'NONE',  ( 0.000000000000000000, 0.000000000000000000, 1.000000000000000000 ) ) ;
#3172=ADVANCED_FACE ( 'NONE', ( #26489 ), #25838, .T. ) ;
#3173=AXIS2_PLACEMENT_3D ( 'NONE', #121620, #113095, #92830 ) ;
#3174=VECTOR ( 'NONE', #45511, 1000.000000000000000 ) ;
#3175=CARTESIAN_POINT ( 'NONE',  ( -6.450000000000017941, 12.50000000000000000, -2.576566944158915184 ) ) ;
#3176=DIRECTION ( 'NONE',  ( 0.000000000000000000, 0.000000000000000000, -1.000000000000000000 ) ) ;
#3177=ORIENTED_EDGE ( 'NONE', *, *, #33618, .T. ) ;
#3178=AXIS2_PLACEMENT_3D ( 'NONE', #34185, #119477, #62360 ) ;
#3179=EDGE_CURVE ( 'NONE', #103010, #37632, #5519, .T. ) ;
#3180=DIRECTION ( 'NONE',  ( -0.000000000000000000, -1.000000000000000000, -0.000000000000000000 ) ) ;
#3181=EDGE_CURVE ( 'NONE', #66905, #53623, #78713, .T. ) ;
#3182=FACE_OUTER_BOUND ( 'NONE', #27854, .T. ) ;
#3183=EDGE_LOOP ( 'NONE', ( #31064, #3649 ) ) ;
#3184=CONICAL_SURFACE ( 'NONE', #21976, 0.1000000000000000472, 0.003490658503988666988 ) ;
#3185=AXIS2_PLACEMENT_3D ( 'NONE', #58803, #90164, #78459 ) ;
#3186=VERTEX_POINT ( 'NONE', #6177 ) ;
#3187=ORIENTED_EDGE ( 'NONE', *, *, #69092, .F. ) ;
#3188=ORIENTED_EDGE ( 'NONE', *, *, #119566, .T. ) ;
#3189=DIRECTION ( 'NONE',  ( -4.274815082592931898E-19, -0.9999939076577903929, -0.003490651415223739937 ) ) ;
#3190=EDGE_CURVE ( 'NONE', #90210, #1124, #55934, .T. ) ;
#3191=AXIS2_PLACEMENT_3D ( 'NONE', #54829, #84300, #112485 ) ;
#3192=EDGE_CURVE ( 'NONE', #105778, #128794, #30601, .T. ) ;
#3194=EDGE_CURVE ( 'NONE', #123846, #56415, #9651, .T. ) ;
#3195=DIRECTION ( 'NONE',  ( 0.000000000000000000, 0.000000000000000000, 1.000000000000000000 ) ) ;
#3197=CIRCLE ( 'NONE', #65872, 0.1000000000000002554 ) ;
#3199=ORIENTED_EDGE ( 'NONE', *, *, #101344, .T. ) ;
#3200=EDGE_CURVE ( 'NONE', #28676, #68600, #73321, .T. ) ;
#3201=CARTESIAN_POINT ( 'NONE',  ( -0.2000000000000347888, 12.50000000000000000, 0.3464101615137758494 ) ) ;
#3202=EDGE_LOOP ( 'NONE', ( #2920, #95882 ) ) ;
#3204=CARTESIAN_POINT ( 'NONE',  ( 10.19999999999991402, 2.500000000000000000, 0.2464101615137735679 ) ) ;
#3205=DIRECTION ( 'NONE',  ( 0.000000000000000000, 1.000000000000000000, 0.000000000000000000 ) ) ;
#3206=DIRECTION ( 'NONE',  ( 0.000000000000000000, -0.000000000000000000, 1.000000000000000000 ) ) ;
#3207=EDGE_CURVE ( 'NONE', #46500, #62111, #76554, .T. ) ;
#3208=ORIENTED_EDGE ( 'NONE', *, *, #10125, .F. ) ;
#3209=ORIENTED_EDGE ( 'NONE', *, *, #101429, .T. ) ;
#3210=ORIENTED_EDGE ( 'NONE', *, *, #6742, .F. ) ;
#3211=LINE ( 'NONE', #72593, #63639 ) ;
#3212=DIRECTION ( 'NONE',  ( 0.000000000000000000, 0.000000000000000000, -1.000000000000000000 ) ) ;
#3213=CARTESIAN_POINT ( 'NONE',  ( -8.150000000000014566, 12.50000000000000000, -6.841600689897073373 ) ) ;
#3214=FACE_BOUND ( 'NONE', #48634, .T. ) ;
#3215=DIRECTION ( 'NONE',  ( 0.000000000000000000, -0.000000000000000000, 1.000000000000000000 ) ) ;
#3216=CIRCLE ( 'NONE', #84775, 0.06509327318403745899 ) ;
#3217=CARTESIAN_POINT ( 'NONE',  ( 4.149999999999938183, 2.500000000000000000, 2.165063509461097713 ) ) ;
#3218=DIRECTION ( 'NONE',  ( 0.000000000000000000, 0.000000000000000000, 1.000000000000000000 ) ) ;
#3219=DIRECTION ( 'NONE',  ( 0.000000000000000000, -0.9999939076577903929, 0.003490651415223739937 ) ) ;
#3220=CIRCLE ( 'NONE', #76379, 0.1000000000000000472 ) ;
#3221=CARTESIAN_POINT ( 'NONE',  ( 9.349999999999919709, 2.500000000000000000, 2.511473670974873507 ) ) ;
#3222=DIRECTION ( 'NONE',  ( 0.000000000000000000, -0.000000000000000000, 1.000000000000000000 ) ) ;
#3223=ORIENTED_EDGE ( 'NONE', *, *, #98933, .T. ) ;
#3224=AXIS2_PLACEMENT_3D ( 'NONE', #41557, #22562, #33027 ) ;
#3225=AXIS2_PLACEMENT_3D ( 'NONE', #95306, #24634, #65830 ) ;
#3226=LINE ( 'NONE', #33969, #39176 ) ;
#3227=ORIENTED_EDGE ( 'NONE', *, *, #117370, .F. ) ;
#3228=ORIENTED_EDGE ( 'NONE', *, *, #82126, .F. ) ;
#3229=CARTESIAN_POINT ( 'NONE',  ( -0.8500000000000390576, 12.50000000000000000, -6.560283801567339701 ) ) ;
#3230=CARTESIAN_POINT ( 'NONE',  ( 11.64999999999990798, 12.50000000000000000, -1.472243186433550122 ) ) ;
#3231=FACE_BOUND ( 'NONE', #114809, .T. ) ;
#3232=DIRECTION ( 'NONE',  ( 0.000000000000000000, 0.000000000000000000, -1.000000000000000000 ) ) ;
#3233=AXIS2_PLACEMENT_3D ( 'NONE', #32196, #44570, #22370 ) ;
#3234=EDGE_CURVE ( 'NONE', #108123, #128150, #14120, .T. ) ;
#3235=CONICAL_SURFACE ( 'NONE', #32500, 0.1000000000000000472, 0.003490658503988666988 ) ;
#3236=ORIENTED_EDGE ( 'NONE', *, *, #104536, .F. ) ;
#3237=CARTESIAN_POINT ( 'NONE',  ( 76.40063402955621541, 3.742348971392434720, 5.987205606707019179 ) ) ;
#3238=CARTESIAN_POINT ( 'NONE',  ( 12.94999999999990337, 12.50000000000000000, 2.230156782645134950 ) ) ;
#3239=EDGE_LOOP ( 'NONE', ( #95473, #118055, #106806, #110930 ) ) ;
#3240=PLANE ( 'NONE',  #49084 ) ;
#3241=PLANE ( 'NONE',  #1070 ) ;
#3242=EDGE_CURVE ( 'NONE', #66905, #32401, #48712, .T. ) ;
#3243=AXIS2_PLACEMENT_3D ( 'NONE', #124759, #114922, #6246 ) ;
#3244=CIRCLE ( 'NONE', #128659, 0.06509327318403745899 ) ;
#3245=VERTEX_POINT ( 'NONE', #1521 ) ;
#3246=DIRECTION ( 'NONE',  ( 0.000000000000000000, 0.000000000000000000, -1.000000000000000000 ) ) ;
#3247=DIRECTION ( 'NONE',  ( 0.000000000000000000, 0.000000000000000000, 1.000000000000000000 ) ) ;
#3248=VERTEX_POINT ( 'NONE', #39559 ) ;
#3249=CARTESIAN_POINT ( 'NONE',  ( -7.700000000000016165, 2.500000000000000000, 0.4464101615137735513 ) ) ;
#3250=FACE_OUTER_BOUND ( 'NONE', #34596, .T. ) ;
#3251=DIRECTION ( 'NONE',  ( -0.000000000000000000, -1.000000000000000000, -0.000000000000000000 ) ) ;
#3252=VERTEX_POINT ( 'NONE', #110830 ) ;
#3253=ORIENTED_EDGE ( 'NONE', *, *, #121232, .T. ) ;
#3254=DIRECTION ( 'NONE',  ( 0.000000000000000000, 0.000000000000000000, 1.000000000000000000 ) ) ;
#3255=VECTOR ( 'NONE', #99409, 1000.000000000000000 ) ;
#3256=VERTEX_POINT ( 'NONE', #61098 ) ;
#3257=CARTESIAN_POINT ( 'NONE',  ( 7.499999999999961808, 2.500000000000000000, -4.330127018922201643 ) ) ;
#3258=DIRECTION ( 'NONE',  ( 0.000000000000000000, 0.000000000000000000, 1.000000000000000000 ) ) ;
#3259=AXIS2_PLACEMENT_3D ( 'NONE', #22590, #93245, #23862 ) ;
#3260=EDGE_LOOP ( 'NONE', ( #11597, #49169, #79485, #33805 ) ) ;
#3261=CIRCLE ( 'NONE', #118266, 0.06509327318403745899 ) ;
#3262=DIRECTION ( 'NONE',  ( 0.000000000000000000, 0.000000000000000000, 1.000000000000000000 ) ) ;
#3263=CARTESIAN_POINT ( 'NONE',  ( 8.949999999999919353, 2.500000000000000000, -6.148780366869526226 ) ) ;
#3264=DIRECTION ( 'NONE',  ( 0.000000000000000000, 0.000000000000000000, 1.000000000000000000 ) ) ;
#3265=CARTESIAN_POINT ( 'NONE',  ( 11.69999999999990514, 12.50000000000000000, -0.06509327318403970719 ) ) ;
#3266=CARTESIAN_POINT ( 'NONE',  ( 6.699999999999928235, 12.50000000000000000, 0.06509327318403515528 ) ) ;
#3267=EDGE_LOOP ( 'NONE', ( #60453, #36787 ) ) ;
#3268=ADVANCED_FACE ( 'NONE', ( #59842 ), #85140, .T. ) ;
#3269=ORIENTED_EDGE ( 'NONE', *, *, #78576, .T. ) ;
#3270=FACE_OUTER_BOUND ( 'NONE', #73156, .T. ) ;
#3271=ORIENTED_EDGE ( 'NONE', *, *, #84429, .F. ) ;
#3272=CARTESIAN_POINT ( 'NONE',  ( -9.550000000000006040, 2.500000000000000000, -2.065063509461102065 ) ) ;
#3273=ORIENTED_EDGE ( 'NONE', *, *, #8608, .T. ) ;
#3274=ORIENTED_EDGE ( 'NONE', *, *, #57367, .T. ) ;
#3275=ORIENTED_EDGE ( 'NONE', *, *, #29635, .T. ) ;
#3276=CARTESIAN_POINT ( 'NONE',  ( -0.2000000000000404232, 2.500000000000000000, 3.983716857408420964 ) ) ;
#3277=AXIS2_PLACEMENT_3D ( 'NONE', #31653, #10079, #71568 ) ;
#3278=PLANE ( 'NONE',  #6707 ) ;
#3279=EDGE_CURVE ( 'NONE', #44934, #5550, #68415, .T. ) ;
#3280=PLANE ( 'NONE',  #89438 ) ;
#3281=VECTOR ( 'NONE', #67002, 1000.000000000000000 ) ;
#3282=CARTESIAN_POINT ( 'NONE',  ( -2.300000000000033573, 2.500000000000000000, 0.3464101615137735735 ) ) ;
#3283=CARTESIAN_POINT ( 'NONE',  ( -10.65000000000000213, 12.50000000000000000, 6.148780366869520009 ) ) ;
#3284=DIRECTION ( 'NONE',  ( 0.000000000000000000, 1.000000000000000000, 0.000000000000000000 ) ) ;
#3285=CIRCLE ( 'NONE', #53466, 0.1000000000000002554 ) ;
#3286=DIRECTION ( 'NONE',  ( -4.274815082592931898E-19, -0.9999939076577903929, -0.003490651415223739937 ) ) ;
#3287=CARTESIAN_POINT ( 'NONE',  ( -5.450000000000023270, 2.500000000000000000, -6.395190528383301931 ) ) ;
#3288=ADVANCED_FACE ( 'NONE', ( #78825 ), #87288, .T. ) ;
#3289=EDGE_CURVE ( 'NONE', #79919, #64213, #9935, .T. ) ;
#3291=EDGE_LOOP ( 'NONE', ( #19664, #66763, #117659, #25180 ) ) ;
#3292=EDGE_CURVE ( 'NONE', #25992, #65903, #30888, .T. ) ;
#3293=DIRECTION ( 'NONE',  ( 0.000000000000000000, -0.000000000000000000, 1.000000000000000000 ) ) ;
#3294=VERTEX_POINT ( 'NONE', #23582 ) ;
#3295=VERTEX_POINT ( 'NONE', #24236 ) ;
#3296=ADVANCED_FACE ( 'NONE', ( #113913 ), #93558, .T. ) ;
#3297=FACE_OUTER_BOUND ( 'NONE', #59393, .T. ) ;
#3298=DIRECTION ( 'NONE',  ( 0.000000000000000000, 1.000000000000000000, 0.000000000000000000 ) ) ;
#3299=CARTESIAN_POINT ( 'NONE',  ( 11.89999999999990443, 2.500000000000000000, -0.3464101615137782364 ) ) ;
#3300=FACE_OUTER_BOUND ( 'NONE', #67755, .T. ) ;
#3301=CARTESIAN_POINT ( 'NONE',  ( 8.949999999999915801, 2.500000000000000000, 6.741600689897071952 ) ) ;
#3302=CARTESIAN_POINT ( 'NONE',  ( 3.099999999999945022, 2.500000000000000000, -4.676537180435978769 ) ) ;
#3303=LINE ( 'NONE', #44509, #82355 ) ;
#3304=ORIENTED_EDGE ( 'NONE', *, *, #31227, .T. ) ;
#3305=AXIS2_PLACEMENT_3D ( 'NONE', #96929, #7249, #47204 ) ;
#3306=CONICAL_SURFACE ( 'NONE', #61904, 0.1000000000000002554, 0.003490658503988666988 ) ;
#3307=AXIS2_PLACEMENT_3D ( 'NONE', #51382, #91282, #41560 ) ;
#3308=CARTESIAN_POINT ( 'NONE',  ( -9.400000000000007461, 2.500000000000000000, 0.3464101615137735735 ) ) ;
#3310=VERTEX_POINT ( 'NONE', #45173 ) ;
#3311=AXIS2_PLACEMENT_3D ( 'NONE', #15755, #46508, #5925 ) ;
#3312=ORIENTED_EDGE ( 'NONE', *, *, #13815, .T. ) ;
#3314=DIRECTION ( 'NONE',  ( 0.000000000000000000, 0.000000000000000000, -1.000000000000000000 ) ) ;
#3315=DIRECTION ( 'NONE',  ( 0.000000000000000000, 1.000000000000000000, 0.000000000000000000 ) ) ;
#3316=AXIS2_PLACEMENT_3D ( 'NONE', #100120, #81130, #29447 ) ;
#3317=DIRECTION ( 'NONE',  ( 0.000000000000000000, 0.000000000000000000, -1.000000000000000000 ) ) ;
#3318=DIRECTION ( 'NONE',  ( 0.000000000000000000, 0.000000000000000000, 1.000000000000000000 ) ) ;
#3319=CONICAL_SURFACE ( 'NONE', #76487, 0.1000000000000000056, 0.003490658503988666988 ) ;
#3321=DIRECTION ( 'NONE',  ( 0.000000000000000000, 1.000000000000000000, 0.000000000000000000 ) ) ;
#3322=ORIENTED_EDGE ( 'NONE', *, *, #48692, .T. ) ;
#3323=DIRECTION ( 'NONE',  ( 0.000000000000000000, 0.000000000000000000, 1.000000000000000000 ) ) ;
#3324=DIRECTION ( 'NONE',  ( 0.000000000000000000, 0.000000000000000000, -1.000000000000000000 ) ) ;
#3325=CARTESIAN_POINT ( 'NONE',  ( -9.150000000000005684, 2.500000000000000000, 7.088010851410848190 ) ) ;
#3326=CARTESIAN_POINT ( 'NONE',  ( -2.900000000000029221, 2.500000000000000000, -4.330127018922201643 ) ) ;
#3327=EDGE_LOOP ( 'NONE', ( #24274, #100808 ) ) ;
#3328=AXIS2_PLACEMENT_3D ( 'NONE', #73554, #113487, #123947 ) ;
#3329=CIRCLE ( 'NONE', #86945, 0.1000000000000002554 ) ;
#3330=ORIENTED_EDGE ( 'NONE', *, *, #128664, .T. ) ;
#3331=VERTEX_POINT ( 'NONE', #56263 ) ;
#3332=EDGE_CURVE ( 'NONE', #74337, #37904, #82828, .T. ) ;
#3333=CARTESIAN_POINT ( 'NONE',  ( 4.999999999999936939, 12.50000000000000000, -3.702399969078687292 ) ) ;
#3334=EDGE_CURVE ( 'NONE', #129288, #48344, #110009, .T. ) ;
#3335=ADVANCED_FACE ( 'NONE', ( #35350 ), #66078, .T. ) ;
#3337=LINE ( 'NONE', #123728, #92547 ) ;
#3338=CARTESIAN_POINT ( 'NONE',  ( -1.450000000000035039, 2.500000000000000000, -6.941600689897077459 ) ) ;
#3339=ADVANCED_FACE ( 'NONE', ( #24879 ), #89359, .T. ) ;
#3341=DIRECTION ( 'NONE',  ( -4.274815082592931898E-19, -0.9999939076577903929, -0.003490651415223739937 ) ) ;
#3342=DIRECTION ( 'NONE',  ( 0.000000000000000000, 0.000000000000000000, -1.000000000000000000 ) ) ;
#3343=LINE ( 'NONE', #54370, #62995 ) ;
#3344=CARTESIAN_POINT ( 'NONE',  ( 8.149999999999920419, 12.50000000000000000, 6.213873640053559022 ) ) ;
#3345=EDGE_CURVE ( 'NONE', #112688, #120493, #76845, .T. ) ;
#3346=EDGE_CURVE ( 'NONE', #39693, #3135, #108131, .T. ) ;
#3347=CIRCLE ( 'NONE', #99504, 0.06509327318403745899 ) ;
#3348=CARTESIAN_POINT ( 'NONE',  ( 4.599999999999936584, 12.50000000000000000, 3.637306695894644726 ) ) ;
#3349=AXIS2_PLACEMENT_3D ( 'NONE', #98292, #89769, #78685 ) ;
#3350=ORIENTED_EDGE ( 'NONE', *, *, #72062, .F. ) ;
#3351=ORIENTED_EDGE ( 'NONE', *, *, #38316, .F. ) ;
#3353=CARTESIAN_POINT ( 'NONE',  ( -0.8500000000000382805, 2.500000000000000000, -1.472243186433550122 ) ) ;
#3354=DIRECTION ( 'NONE',  ( 0.000000000000000000, 0.000000000000000000, 1.000000000000000000 ) ) ;
#3355=FACE_OUTER_BOUND ( 'NONE', #62813, .T. ) ;
#3356=CIRCLE ( 'NONE', #108096, 0.06509327318403745899 ) ;
#3357=DIRECTION ( 'NONE',  ( -0.000000000000000000, 1.000000000000000000, -0.000000000000000000 ) ) ;
#3358=EDGE_LOOP ( 'NONE', ( #37425, #31143, #33559, #129211 ) ) ;
#3359=VERTEX_POINT ( 'NONE', #84444 ) ;
#3360=CARTESIAN_POINT ( 'NONE',  ( -6.650000000000018119, 12.50000000000000000, -6.495190528383302464 ) ) ;
#3361=CARTESIAN_POINT ( 'NONE',  ( 3.149999999999942624, 12.50000000000000000, 6.841600689897072485 ) ) ;
#3362=DIRECTION ( 'NONE',  ( -0.000000000000000000, -1.000000000000000000, -0.000000000000000000 ) ) ;
#3363=FACE_OUTER_BOUND ( 'NONE', #99898, .T. ) ;
#3365=VERTEX_POINT ( 'NONE', #6483 ) ;
#3366=DIRECTION ( 'NONE',  ( 0.000000000000000000, 0.000000000000000000, 1.000000000000000000 ) ) ;
#3367=CONICAL_SURFACE ( 'NONE', #34780, 0.09999999999999982514, 0.003490658503988666988 ) ;
#3368=FACE_OUTER_BOUND ( 'NONE', #92228, .T. ) ;
#3369=ORIENTED_EDGE ( 'NONE', *, *, #104376, .T. ) ;
#3370=CARTESIAN_POINT ( 'NONE',  ( 12.09999999999990195, 2.500000000000000000, -0.5928203230275541635 ) ) ;
#3371=ORIENTED_EDGE ( 'NONE', *, *, #112669, .F. ) ;
#3372=DIRECTION ( 'NONE',  ( 0.000000000000000000, 0.000000000000000000, 1.000000000000000000 ) ) ;
#3373=ORIENTED_EDGE ( 'NONE', *, *, #128523, .T. ) ;
#3374=DIRECTION ( 'NONE',  ( 0.000000000000000000, 1.000000000000000000, 0.000000000000000000 ) ) ;
#3375=CARTESIAN_POINT ( 'NONE',  ( 8.099999999999923261, 2.500000000000000000, 4.676537180435972552 ) ) ;
#3376=ORIENTED_EDGE ( 'NONE', *, *, #118536, .F. ) ;
#3377=ORIENTED_EDGE ( 'NONE', *, *, #95198, .T. ) ;
#3382=EDGE_CURVE ( 'NONE', #68225, #79959, #32949, .T. ) ;
#3383=AXIS2_PLACEMENT_3D ( 'NONE', #7151, #39241, #49693 ) ;
#3384=DIRECTION ( 'NONE',  ( 0.000000000000000000, 1.000000000000000000, 0.000000000000000000 ) ) ;
#3385=DIRECTION ( 'NONE',  ( 0.000000000000000000, 0.000000000000000000, -1.000000000000000000 ) ) ;
#3386=EDGE_CURVE ( 'NONE', #127025, #98360, #116247, .T. ) ;
#3387=CARTESIAN_POINT ( 'NONE',  ( 1.649999999999951505, 12.50000000000000000, 1.472243186433545459 ) ) ;
#3388=CONICAL_SURFACE ( 'NONE', #57779, 0.1000000000000000472, 0.003490658503988666988 ) ;
#3389=CARTESIAN_POINT ( 'NONE',  ( -9.600000000000008527, 2.500000000000000000, -0.1000000000000023925 ) ) ;
#3390=AXIS2_PLACEMENT_3D ( 'NONE', #55704, #85802, #45254 ) ;
#3391=AXIS2_PLACEMENT_3D ( 'NONE', #88541, #49939, #47994 ) ;
#3392=EDGE_LOOP ( 'NONE', ( #67767, #117672 ) ) ;
#3393=AXIS2_PLACEMENT_3D ( 'NONE', #23661, #63591, #103513 ) ;
#3394=VERTEX_POINT ( 'NONE', #14393 ) ;
#3395=DIRECTION ( 'NONE',  ( 0.000000000000000000, 0.000000000000000000, -1.000000000000000000 ) ) ;
#3396=ORIENTED_EDGE ( 'NONE', *, *, #93946, .T. ) ;
#3397=LINE ( 'NONE', #44614, #60100 ) ;
#3398=DIRECTION ( 'NONE',  ( 0.000000000000000000, 0.000000000000000000, 1.000000000000000000 ) ) ;
#3399=CARTESIAN_POINT ( 'NONE',  ( -6.249999999999981348, 12.50000000000000000, 2.099970236277060032 ) ) ;
#3400=VERTEX_POINT ( 'NONE', #105373 ) ;
#3401=EDGE_LOOP ( 'NONE', ( #97852, #102026 ) ) ;
#3402=FACE_BOUND ( 'NONE', #64250, .T. ) ;
#3403=ORIENTED_EDGE ( 'NONE', *, *, #97045, .T. ) ;
#3404=DIRECTION ( 'NONE',  ( 0.000000000000000000, 0.000000000000000000, -1.000000000000000000 ) ) ;
#3405=CARTESIAN_POINT ( 'NONE',  ( -8.150000000000014566, 2.500000000000000000, -6.148780366869520897 ) ) ;
#3406=AXIS2_PLACEMENT_3D ( 'NONE', #54867, #94806, #86909 ) ;
#3407=DIRECTION ( 'NONE',  ( -4.274815082592931898E-19, -0.9999939076577903929, -0.003490651415223739937 ) ) ;
#3408=CARTESIAN_POINT ( 'NONE',  ( -3.350000000000032507, 12.50000000000000000, -6.560283801567339701 ) ) ;
#3409=DIRECTION ( 'NONE',  ( -0.000000000000000000, 1.000000000000000000, -0.000000000000000000 ) ) ;
#3410=AXIS2_PLACEMENT_3D ( 'NONE', #12274, #63973, #4370 ) ;
#3411=VECTOR ( 'NONE', #65548, 1000.000000000000000 ) ;
#3412=CARTESIAN_POINT ( 'NONE',  ( 9.599999999999914380, 2.500000000000000000, 4.230127018922196669 ) ) ;
#3413=CARTESIAN_POINT ( 'NONE',  ( -2.499999999999996003, 2.500000000000000000, -4.330127018922201643 ) ) ;
#3414=FACE_OUTER_BOUND ( 'NONE', #56837, .T. ) ;
#3415=CARTESIAN_POINT ( 'NONE',  ( 10.39999999999990976, 12.50000000000000000, -4.330127018922201643 ) ) ;
#3416=DIRECTION ( 'NONE',  ( 0.000000000000000000, 0.000000000000000000, 1.000000000000000000 ) ) ;
#3417=CARTESIAN_POINT ( 'NONE',  ( -2.100000000000034728, 2.500000000000000000, 4.330127018922196314 ) ) ;
#3418=ORIENTED_EDGE ( 'NONE', *, *, #79445, .T. ) ;
#3419=ORIENTED_EDGE ( 'NONE', *, *, #16024, .F. ) ;
#3420=ORIENTED_EDGE ( 'NONE', *, *, #31519, .T. ) ;
#3421=CARTESIAN_POINT ( 'NONE',  ( -4.600000000000024514, 2.500000000000000000, 3.537306695894645081 ) ) ;
#3423=LINE ( 'NONE', #23718, #56991 ) ;
#3424=ORIENTED_EDGE ( 'NONE', *, *, #33121, .F. ) ;
#3425=ORIENTED_EDGE ( 'NONE', *, *, #99659, .F. ) ;
#3427=EDGE_CURVE ( 'NONE', #59532, #121105, #49385, .T. ) ;
#3428=DIRECTION ( 'NONE',  ( 0.000000000000000000, 1.000000000000000000, 0.000000000000000000 ) ) ;
#3430=DIRECTION ( 'NONE',  ( 0.000000000000000000, 1.000000000000000000, 0.000000000000000000 ) ) ;
#3431=CARTESIAN_POINT ( 'NONE',  ( -10.85000000000000142, 2.500000000000000000, -1.472243186433546125 ) ) ;
#3432=CARTESIAN_POINT ( 'NONE',  ( -10.85000000000000142, 2.500000000000000000, -7.188010851410850499 ) ) ;
#3433=DIRECTION ( 'NONE',  ( -0.000000000000000000, 1.000000000000000000, -0.000000000000000000 ) ) ;
#3434=EDGE_CURVE ( 'NONE', #17761, #23241, #124867, .T. ) ;
#3435=VERTEX_POINT ( 'NONE', #93618 ) ;
#3436=EDGE_CURVE ( 'NONE', #27815, #11046, #99831, .T. ) ;
#3437=CARTESIAN_POINT ( 'NONE',  ( -13.09999999999999254, 12.50000000000000000, -4.048810130592460865 ) ) ;
#3438=EDGE_LOOP ( 'NONE', ( #36438, #19297 ) ) ;
#3439=VECTOR ( 'NONE', #96293, 1000.000000000000000 ) ;
#3440=EDGE_LOOP ( 'NONE', ( #39912, #43577, #78100, #124381 ) ) ;
#3441=ORIENTED_EDGE ( 'NONE', *, *, #101429, .F. ) ;
#3442=AXIS2_PLACEMENT_3D ( 'NONE', #37941, #117763, #7176 ) ;
#3443=EDGE_CURVE ( 'NONE', #45043, #117937, #4553, .T. ) ;
#3444=FACE_OUTER_BOUND ( 'NONE', #77319, .T. ) ;
#3445=EDGE_CURVE ( 'NONE', #83081, #46534, #122522, .T. ) ;
#3446=ADVANCED_FACE ( 'NONE', ( #45816 ), #85718, .T. ) ;
#3447=ORIENTED_EDGE ( 'NONE', *, *, #3382, .F. ) ;
#3448=EDGE_LOOP ( 'NONE', ( #37278, #76317, #63856, #57143 ) ) ;
#3449=EDGE_CURVE ( 'NONE', #127462, #21944, #87648, .T. ) ;
#3450=EDGE_CURVE ( 'NONE', #97893, #38892, #99550, .T. ) ;
#3451=EDGE_LOOP ( 'NONE', ( #102852, #27685 ) ) ;
#3453=VECTOR ( 'NONE', #10303, 1000.000000000000000 ) ;
#3454=CARTESIAN_POINT ( 'NONE',  ( 14.79999999999989413, 2.500000000000000000, -0.3464101615137782364 ) ) ;
#3455=CARTESIAN_POINT ( 'NONE',  ( -3.950000000000025491, 12.50000000000000000, 6.148780366869520897 ) ) ;
#3456=DIRECTION ( 'NONE',  ( -0.000000000000000000, -1.000000000000000000, -0.000000000000000000 ) ) ;
#3457=DIRECTION ( 'NONE',  ( -4.274815082592931898E-19, -0.9999939076577903929, -0.003490651415223739937 ) ) ;
#3458=CARTESIAN_POINT ( 'NONE',  ( 2.500000000000002220, 1.499999999999999334, 10.00000000000000178 ) ) ;
#3459=EDGE_CURVE ( 'NONE', #43141, #22334, #5714, .T. ) ;
#3460=PLANE ( 'NONE',  #124454 ) ;
#3461=AXIS2_PLACEMENT_3D ( 'NONE', #38769, #80604, #101528 ) ;
#3462=CIRCLE ( 'NONE', #105866, 0.09999999999999999167 ) ;
#3463=ORIENTED_EDGE ( 'NONE', *, *, #1351, .T. ) ;
#3464=CARTESIAN_POINT ( 'NONE',  ( -12.89999999999999147, 2.500000000000000000, -5.122947341949751987 ) ) ;
#3465=AXIS2_PLACEMENT_3D ( 'NONE', #68798, #59659, #99562 ) ;
#3466=ORIENTED_EDGE ( 'NONE', *, *, #104129, .F. ) ;
#3468=ORIENTED_EDGE ( 'NONE', *, *, #15008, .T. ) ;
#3469=VERTEX_POINT ( 'NONE', #127591 ) ;
#3470=DIRECTION ( 'NONE',  ( 0.000000000000000000, -0.9999939076577903929, 0.003490651415223739937 ) ) ;
#3471=FACE_OUTER_BOUND ( 'NONE', #18024, .T. ) ;
#3472=DIRECTION ( 'NONE',  ( 0.000000000000000000, -0.9999939076577903929, 0.003490651415223739937 ) ) ;
#3473=ORIENTED_EDGE ( 'NONE', *, *, #99194, .F. ) ;
#3474=ORIENTED_EDGE ( 'NONE', *, *, #52438, .F. ) ;
#3475=DIRECTION ( 'NONE',  ( 0.000000000000000000, 0.000000000000000000, 1.000000000000000000 ) ) ;
#3476=DIRECTION ( 'NONE',  ( 0.000000000000000000, 1.000000000000000000, 0.000000000000000000 ) ) ;
#3477=DIRECTION ( 'NONE',  ( -0.000000000000000000, -1.000000000000000000, -0.000000000000000000 ) ) ;
#3478=CIRCLE ( 'NONE', #101687, 0.1000000000000000472 ) ;
#3479=CARTESIAN_POINT ( 'NONE',  ( 0.1999999999999576006, 2.500000000000000000, -4.776537180435978414 ) ) ;
#3480=AXIS2_PLACEMENT_3D ( 'NONE', #19845, #40123, #8698 ) ;
#3481=DIRECTION ( 'NONE',  ( 0.000000000000000000, 1.000000000000000000, 0.000000000000000000 ) ) ;
#3482=ORIENTED_EDGE ( 'NONE', *, *, #121427, .F. ) ;
#3483=VECTOR ( 'NONE', #75617, 1000.000000000000000 ) ;
#3484=DIRECTION ( 'NONE',  ( 0.000000000000000000, 0.000000000000000000, -1.000000000000000000 ) ) ;
#3485=ADVANCED_FACE ( 'NONE', ( #116465 ), #45461, .T. ) ;
#3486=EDGE_CURVE ( 'NONE', #39867, #75029, #66520, .T. ) ;
#3487=AXIS2_PLACEMENT_3D ( 'NONE', #88045, #95324, #76972 ) ;
#3488=EDGE_CURVE ( 'NONE', #1760, #96273, #24776, .T. ) ;
#3489=ORIENTED_EDGE ( 'NONE', *, *, #86026, .F. ) ;
#3490=CIRCLE ( 'NONE', #22379, 0.06509327318403745899 ) ;
#3491=PLANE ( 'NONE',  #77873 ) ;
#3492=CARTESIAN_POINT ( 'NONE',  ( -8.350000000000008527, 2.500000000000000000, 7.188010851410848723 ) ) ;
#3493=AXIS2_PLACEMENT_3D ( 'NONE', #86272, #56807, #96740 ) ;
#3494=EDGE_CURVE ( 'NONE', #24755, #48591, #64470, .T. ) ;
#3496=DIRECTION ( 'NONE',  ( 0.000000000000000000, -0.9999939076577903929, 0.003490651415223739937 ) ) ;
#3497=VECTOR ( 'NONE', #55590, 1000.000000000000000 ) ;
#3498=DIRECTION ( 'NONE',  ( 0.000000000000000000, 1.000000000000000000, 0.000000000000000000 ) ) ;
#3499=EDGE_CURVE ( 'NONE', #7675, #58472, #107946, .T. ) ;
#3500=CARTESIAN_POINT ( 'NONE',  ( 5.449999999999937117, 2.500000000000000000, -6.495190528383302464 ) ) ;
#3501=DIRECTION ( 'NONE',  ( 0.000000000000000000, 1.000000000000000000, 0.000000000000000000 ) ) ;
#3502=ORIENTED_EDGE ( 'NONE', *, *, #121383, .F. ) ;
#3503=CONICAL_SURFACE ( 'NONE', #22306, 0.1000000000000002554, 0.003490658503988666988 ) ;
#3504=EDGE_CURVE ( 'NONE', #37160, #18098, #14287, .T. ) ;
#3505=EDGE_CURVE ( 'NONE', #23967, #2289, #122975, .T. ) ;
#3506=FACE_OUTER_BOUND ( 'NONE', #122936, .T. ) ;
#3507=CIRCLE ( 'NONE', #20233, 0.1000000000000002554 ) ;
#3508=CIRCLE ( 'NONE', #51636, 0.06509327318403745899 ) ;
#3509=EDGE_CURVE ( 'NONE', #18231, #108081, #10100, .T. ) ;
#3510=DIRECTION ( 'NONE',  ( 0.000000000000000000, 0.000000000000000000, 1.000000000000000000 ) ) ;
#3511=DIRECTION ( 'NONE',  ( -0.000000000000000000, 1.000000000000000000, -0.000000000000000000 ) ) ;
#3512=EDGE_LOOP ( 'NONE', ( #121905, #118922, #119382, #22083 ) ) ;
#3513=EDGE_CURVE ( 'NONE', #67817, #57536, #39376, .T. ) ;
#3514=CARTESIAN_POINT ( 'NONE',  ( -5.600000000000020073, 12.50000000000000000, 0.3464101615137736845 ) ) ;
#3515=ORIENTED_EDGE ( 'NONE', *, *, #7885, .T. ) ;
#3516=LINE ( 'NONE', #24444, #34309 ) ;
#3517=ORIENTED_EDGE ( 'NONE', *, *, #98379, .T. ) ;
#3518=CARTESIAN_POINT ( 'NONE',  ( 17.17161331426590820, -0.4678040054246333512, -5.513957101014161921 ) ) ;
#3519=CARTESIAN_POINT ( 'NONE',  ( -8.749999999999975131, 2.500000000000000000, -2.065063509461102065 ) ) ;
#3520=VECTOR ( 'NONE', #97276, 1000.000000000000000 ) ;
#3522=VERTEX_POINT ( 'NONE', #9749 ) ;
#3523=FACE_OUTER_BOUND ( 'NONE', #122181, .T. ) ;
#3525=ADVANCED_FACE ( 'NONE', ( #128250 ), #67340, .T. ) ;
#3527=VECTOR ( 'NONE', #69254, 1000.000000000000000 ) ;
#3528=VERTEX_POINT ( 'NONE', #39874 ) ;
#3529=AXIS2_PLACEMENT_3D ( 'NONE', #14265, #36984, #54210 ) ;
#3530=ORIENTED_EDGE ( 'NONE', *, *, #60954, .T. ) ;
#3531=CARTESIAN_POINT ( 'NONE',  ( 4.149999999999938183, 2.500000000000000000, 7.188010851410848723 ) ) ;
#3532=DIRECTION ( 'NONE',  ( 0.000000000000000000, -0.000000000000000000, 1.000000000000000000 ) ) ;
#3533=DIRECTION ( 'NONE',  ( 0.000000000000000000, 1.000000000000000000, 0.000000000000000000 ) ) ;
#3534=ORIENTED_EDGE ( 'NONE', *, *, #22511, .T. ) ;
#3535=CARTESIAN_POINT ( 'NONE',  ( -10.00000000000000533, 12.50000000000000000, 0.6928203230275494784 ) ) ;
#3538=VECTOR ( 'NONE', #68697, 1000.000000000000000 ) ;
#3539=AXIS2_PLACEMENT_3D ( 'NONE', #112059, #32871, #120585 ) ;
#3540=DIRECTION ( 'NONE',  ( -0.000000000000000000, -1.000000000000000000, -0.000000000000000000 ) ) ;
#3541=CARTESIAN_POINT ( 'NONE',  ( 12.49999999999990408, 2.500000000000000000, -3.637306695894650055 ) ) ;
#3542=EDGE_CURVE ( 'NONE', #80322, #120641, #114641, .T. ) ;
#3543=PLANE ( 'NONE',  #82141 ) ;
#3544=DIRECTION ( 'NONE',  ( 0.000000000000000000, -0.000000000000000000, 1.000000000000000000 ) ) ;
#3545=DIRECTION ( 'NONE',  ( 0.000000000000000000, 0.000000000000000000, 1.000000000000000000 ) ) ;
#3546=CARTESIAN_POINT ( 'NONE',  ( 4.549999999999939426, 12.50000000000000000, -6.495190528383302464 ) ) ;
#3547=CARTESIAN_POINT ( 'NONE',  ( 4.999999999999969802, 12.50000000000000000, 4.330127018922196314 ) ) ;
#3548=CONICAL_SURFACE ( 'NONE', #18117, 0.09999999999999982514, 0.003490658503988666988 ) ;
#3549=VECTOR ( 'NONE', #2247, 1000.000000000000000 ) ;
#3550=ORIENTED_EDGE ( 'NONE', *, *, #28438, .T. ) ;
#3551=ORIENTED_EDGE ( 'NONE', *, *, #59969, .T. ) ;
#3552=ORIENTED_EDGE ( 'NONE', *, *, #80457, .F. ) ;
#3553=ORIENTED_EDGE ( 'NONE', *, *, #8226, .F. ) ;
#3555=DIRECTION ( 'NONE',  ( 0.000000000000000000, -0.9999939076577903929, 0.003490651415223739937 ) ) ;
#3556=CARTESIAN_POINT ( 'NONE',  ( 4.599999999999936584, 2.500000000000000000, 4.230127018922196669 ) ) ;
#3557=ORIENTED_EDGE ( 'NONE', *, *, #95557, .T. ) ;
#3558=EDGE_CURVE ( 'NONE', #127371, #111304, #79150, .T. ) ;
#3559=FACE_BOUND ( 'NONE', #123016, .T. ) ;
#3560=DIRECTION ( 'NONE',  ( -0.000000000000000000, 1.000000000000000000, -0.000000000000000000 ) ) ;
#3561=FACE_OUTER_BOUND ( 'NONE', #121386, .T. ) ;
#3562=CARTESIAN_POINT ( 'NONE',  ( 8.949999999999915801, 12.50000000000000000, -1.818653347947326138 ) ) ;
#3563=DIRECTION ( 'NONE',  ( -0.000000000000000000, -1.000000000000000000, -0.000000000000000000 ) ) ;
#3564=DIRECTION ( 'NONE',  ( 0.000000000000000000, 0.000000000000000000, -1.000000000000000000 ) ) ;
#3565=DIRECTION ( 'NONE',  ( 0.000000000000000000, 1.000000000000000000, 0.000000000000000000 ) ) ;
#3566=PLANE ( 'NONE',  #68491 ) ;
#3567=CARTESIAN_POINT ( 'NONE',  ( -3.350000000000031619, 12.50000000000000000, -7.188010851410854052 ) ) ;
#3568=CARTESIAN_POINT ( 'NONE',  ( -0.6000000000000383915, 2.500000000000000000, -4.776537180435977525 ) ) ;
#3569=CONICAL_SURFACE ( 'NONE', #91304, 0.1000000000000002554, 0.003490658503988666988 ) ;
#3570=AXIS2_PLACEMENT_3D ( 'NONE', #63472, #1315, #32740 ) ;
#3571=VECTOR ( 'NONE', #20329, 1000.000000000000000 ) ;
#3572=EDGE_LOOP ( 'NONE', ( #126726, #6009 ) ) ;
#3573=ORIENTED_EDGE ( 'NONE', *, *, #18938, .F. ) ;
#3574=CONICAL_SURFACE ( 'NONE', #103929, 0.1000000000000002554, 0.003490658503988666988 ) ;
#3575=VERTEX_POINT ( 'NONE', #48384 ) ;
#3576=ORIENTED_EDGE ( 'NONE', *, *, #104827, .T. ) ;
#3577=ORIENTED_EDGE ( 'NONE', *, *, #75925, .F. ) ;
#3578=ORIENTED_EDGE ( 'NONE', *, *, #74897, .F. ) ;
#3579=DIRECTION ( 'NONE',  ( 0.000000000000000000, 0.000000000000000000, 1.000000000000000000 ) ) ;
#3580=ORIENTED_EDGE ( 'NONE', *, *, #45192, .F. ) ;
#3581=CIRCLE ( 'NONE', #105986, 0.06509327318403745899 ) ;
#3582=EDGE_LOOP ( 'NONE', ( #58539, #96317, #11080, #105455 ) ) ;
#3583=CIRCLE ( 'NONE', #112340, 0.1000000000000002554 ) ;
#3584=CONICAL_SURFACE ( 'NONE', #53667, 0.1000000000000000472, 0.003490658503988666988 ) ;
#3585=EDGE_CURVE ( 'NONE', #69257, #94819, #68675, .T. ) ;
#3586=DIRECTION ( 'NONE',  ( 0.000000000000000000, 1.000000000000000000, 0.000000000000000000 ) ) ;
#3587=CARTESIAN_POINT ( 'NONE',  ( -10.65000000000000391, 2.500000000000000000, -6.841600689897075149 ) ) ;
#3589=EDGE_LOOP ( 'NONE', ( #73522, #101539, #87655, #12064 ) ) ;
#3590=DIRECTION ( 'NONE',  ( -0.000000000000000000, -1.000000000000000000, -0.000000000000000000 ) ) ;
#3591=ADVANCED_FACE ( 'NONE', ( #89600 ), #5872, .T. ) ;
#3592=EDGE_LOOP ( 'NONE', ( #92258, #106785, #77770, #120453 ) ) ;
#3593=CIRCLE ( 'NONE', #95626, 0.1000000000000000472 ) ;
#3594=CIRCLE ( 'NONE', #76758, 0.06509327318403741736 ) ;
#3595=ORIENTED_EDGE ( 'NONE', *, *, #42802, .T. ) ;
#3596=DIRECTION ( 'NONE',  ( 1.000000000000000000, 0.000000000000000000, -0.000000000000000000 ) ) ;
#3597=ADVANCED_FACE ( 'NONE', ( #109219 ), #129550, .T. ) ;
#3598=CARTESIAN_POINT ( 'NONE',  ( -9.600000000000008527, 2.500000000000000000, -2.385244779468109755E-15 ) ) ;
#3599=EDGE_CURVE ( 'NONE', #33854, #88432, #70603, .T. ) ;
#3600=EDGE_CURVE ( 'NONE', #77153, #67249, #16332, .T. ) ;
#3601=EDGE_CURVE ( 'NONE', #28402, #45029, #22171, .T. ) ;
#3602=ORIENTED_EDGE ( 'NONE', *, *, #128653, .T. ) ;
#3603=ORIENTED_EDGE ( 'NONE', *, *, #57412, .F. ) ;
#3604=CARTESIAN_POINT ( 'NONE',  ( 11.44999999999990870, 12.50000000000000000, -1.818653347947326138 ) ) ;
#3605=CARTESIAN_POINT ( 'NONE',  ( -13.29999999999999005, 2.500000000000000000, -4.330127018922198978 ) ) ;
#3606=DIRECTION ( 'NONE',  ( 0.000000000000000000, 0.000000000000000000, 1.000000000000000000 ) ) ;
#3607=DIRECTION ( 'NONE',  ( 0.000000000000000000, 1.000000000000000000, 0.000000000000000000 ) ) ;
#3608=CARTESIAN_POINT ( 'NONE',  ( -8.350000000000013856, 2.500000000000000000, -5.802370205355744659 ) ) ;
#3609=CIRCLE ( 'NONE', #124888, 0.06509327318403745899 ) ;
#3610=EDGE_CURVE ( 'NONE', #117538, #114610, #30045, .T. ) ;
#3611=EDGE_LOOP ( 'NONE', ( #86232, #86347 ) ) ;
#3612=CARTESIAN_POINT ( 'NONE',  ( 11.69999999999990870, 12.50000000000000000, -4.265033745738164406 ) ) ;
#3613=ADVANCED_FACE ( 'NONE', ( #80433 ), #8026, .T. ) ;
#3614=ADVANCED_FACE ( 'NONE', ( #2486 ), #81213, .T. ) ;
#3615=ORIENTED_EDGE ( 'NONE', *, *, #109543, .T. ) ;
#3616=DIRECTION ( 'NONE',  ( 0.000000000000000000, 0.000000000000000000, 1.000000000000000000 ) ) ;
#3617=VERTEX_POINT ( 'NONE', #12317 ) ;
#3618=DIRECTION ( 'NONE',  ( 0.000000000000000000, -0.9999939076577903929, 0.003490651415223739937 ) ) ;
#3619=CARTESIAN_POINT ( 'NONE',  ( 13.74999999999993072, 12.50000000000000000, -2.099970236277064473 ) ) ;
#3620=DIRECTION ( 'NONE',  ( -4.274815082592931898E-19, -0.9999939076577903929, -0.003490651415223739937 ) ) ;
#3621=CARTESIAN_POINT ( 'NONE',  ( 10.39999999999991331, 12.50000000000000000, -2.385244779468109755E-15 ) ) ;
#3622=VERTEX_POINT ( 'NONE', #69965 ) ;
#3624=AXIS2_PLACEMENT_3D ( 'NONE', #119018, #91485, #110482 ) ;
#3625=CARTESIAN_POINT ( 'NONE',  ( 1.249999999999953815, 12.50000000000000000, 1.472243186433545459 ) ) ;
#3626=EDGE_LOOP ( 'NONE', ( #90392, #112551, #68546, #57210 ) ) ;
#3627=VERTEX_POINT ( 'NONE', #90884 ) ;
#3628=ORIENTED_EDGE ( 'NONE', *, *, #49397, .F. ) ;
#3629=CARTESIAN_POINT ( 'NONE',  ( 14.54999999999989235, 2.500000000000000000, -2.165063509461101710 ) ) ;
#3630=CARTESIAN_POINT ( 'NONE',  ( 12.89999999999989733, 12.50000000000000000, -0.06509327318403980434 ) ) ;
#3632=CARTESIAN_POINT ( 'NONE',  ( -17.50000000000000000, 1.500000000000000000, 10.00000000000000178 ) ) ;
#3633=AXIS2_PLACEMENT_3D ( 'NONE', #128285, #78547, #9780 ) ;
#3635=CIRCLE ( 'NONE', #68468, 0.06509327318403745899 ) ;
#3636=CARTESIAN_POINT ( 'NONE',  ( 12.29999999999990123, 2.500000000000000000, 0.3464101615137735735 ) ) ;
#3637=CARTESIAN_POINT ( 'NONE',  ( 11.89999999999990798, 2.500000000000000000, -3.983716857408426293 ) ) ;
#3638=VECTOR ( 'NONE', #125353, 1000.000000000000000 ) ;
#3639=AXIS2_PLACEMENT_3D ( 'NONE', #12384, #42518, #20925 ) ;
#3640=ORIENTED_EDGE ( 'NONE', *, *, #37311, .F. ) ;
#3641=DIRECTION ( 'NONE',  ( 0.000000000000000000, 0.000000000000000000, 1.000000000000000000 ) ) ;
#3642=CIRCLE ( 'NONE', #20376, 0.09999999999999982514 ) ;
#3644=DIRECTION ( 'NONE',  ( 0.000000000000000000, 0.000000000000000000, 1.000000000000000000 ) ) ;
#3645=CARTESIAN_POINT ( 'NONE',  ( 12.49999999999990408, 12.50000000000000000, -3.702399969078687292 ) ) ;
#3646=CARTESIAN_POINT ( 'NONE',  ( 13.74999999999989342, 2.500000000000000000, -1.472243186433550122 ) ) ;
#3647=EDGE_CURVE ( 'NONE', #73941, #33867, #37300, .T. ) ;
#3648=CARTESIAN_POINT ( 'NONE',  ( 6.449999999999930012, 2.500000000000000000, 1.718653347947321386 ) ) ;
#3649=ORIENTED_EDGE ( 'NONE', *, *, #122494, .T. ) ;
#3650=EDGE_CURVE ( 'NONE', #80364, #85528, #76997, .T. ) ;
#3651=ADVANCED_FACE ( 'NONE', ( #109887 ), #41519, .T. ) ;
#3652=CARTESIAN_POINT ( 'NONE',  ( 14.99999999999989164, 2.500000000000000000, 0.5928203230275495006 ) ) ;
#3653=CARTESIAN_POINT ( 'NONE',  ( 12.49999999999993605, 2.500000000000000000, -0.1000000000000022815 ) ) ;
#3654=EDGE_LOOP ( 'NONE', ( #31160, #87146, #118674, #110661 ) ) ;
#3655=VECTOR ( 'NONE', #11620, 1000.000000000000000 ) ;
#3656=AXIS2_PLACEMENT_3D ( 'NONE', #34358, #114819, #71191 ) ;
#3657=VERTEX_POINT ( 'NONE', #60785 ) ;
#3658=EDGE_CURVE ( 'NONE', #18238, #102257, #20570, .T. ) ;
#3659=CARTESIAN_POINT ( 'NONE',  ( 1.249999999999953815, 2.500000000000000000, 1.472243186433545459 ) ) ;
#3660=AXIS2_PLACEMENT_3D ( 'NONE', #23948, #16670, #96522 ) ;
#3661=EDGE_LOOP ( 'NONE', ( #104647, #108613 ) ) ;
#3662=VERTEX_POINT ( 'NONE', #120992 ) ;
#3663=DIRECTION ( 'NONE',  ( 0.000000000000000000, 0.000000000000000000, -1.000000000000000000 ) ) ;
#3664=AXIS2_PLACEMENT_3D ( 'NONE', #73580, #21935, #12092 ) ;
#3665=ORIENTED_EDGE ( 'NONE', *, *, #128331, .T. ) ;
#3666=CARTESIAN_POINT ( 'NONE',  ( 17.84432265422998043, 2.533187527836770148, -5.021315468708433372 ) ) ;
#3668=AXIS2_PLACEMENT_3D ( 'NONE', #67791, #19998, #59938 ) ;
#3669=DIRECTION ( 'NONE',  ( 0.000000000000000000, 1.000000000000000000, 0.000000000000000000 ) ) ;
#3670=EDGE_LOOP ( 'NONE', ( #4354, #86300, #85356, #6712 ) ) ;
#3671=CIRCLE ( 'NONE', #53857, 0.1000000000000000472 ) ;
#3672=CARTESIAN_POINT ( 'NONE',  ( -11.25000000000000178, 2.500000000000000000, -1.472243186433546125 ) ) ;
#3673=CARTESIAN_POINT ( 'NONE',  ( 12.89999999999990088, 2.500000000000000000, -4.430127018922202176 ) ) ;
#3674=ORIENTED_EDGE ( 'NONE', *, *, #120514, .T. ) ;
#3676=CIRCLE ( 'NONE', #106086, 0.1000000000000000472 ) ;
#3677=CARTESIAN_POINT ( 'NONE',  ( 17.34778429999909122, -2.317753570193370027, 4.873671836816545699 ) ) ;
#3678=EDGE_CURVE ( 'NONE', #17419, #41508, #122294, .T. ) ;
#3679=VERTEX_POINT ( 'NONE', #1212 ) ;
#3680=ORIENTED_EDGE ( 'NONE', *, *, #111499, .T. ) ;
#3681=VERTEX_POINT ( 'NONE', #31980 ) ;
#3682=ORIENTED_EDGE ( 'NONE', *, *, #103804, .F. ) ;
#3683=CARTESIAN_POINT ( 'NONE',  ( -13.29999999999999005, 2.500000000000000000, 0.1000000000000018513 ) ) ;
#3684=DIRECTION ( 'NONE',  ( -0.000000000000000000, -1.000000000000000000, -0.000000000000000000 ) ) ;
#3685=CARTESIAN_POINT ( 'NONE',  ( -8.100000000000013856, 12.50000000000000000, -4.676537180435977881 ) ) ;
#3686=FACE_BOUND ( 'NONE', #27157, .T. ) ;
#3687=ORIENTED_EDGE ( 'NONE', *, *, #24270, .F. ) ;
#3689=CARTESIAN_POINT ( 'NONE',  ( -7.499999999999976907, 2.500000000000000000, 4.330127018922196314 ) ) ;
#3690=LINE ( 'NONE', #124105, #43775 ) ;
#3691=EDGE_CURVE ( 'NONE', #91731, #88053, #12949, .T. ) ;
#3692=FACE_OUTER_BOUND ( 'NONE', #84321, .T. ) ;
#3693=CARTESIAN_POINT ( 'NONE',  ( 13.34999999999990017, 2.500000000000000000, 1.372243186433545370 ) ) ;
#3694=CIRCLE ( 'NONE', #76867, 0.06509327318403745899 ) ;
#3695=DIRECTION ( 'NONE',  ( -0.000000000000000000, -1.000000000000000000, -0.000000000000000000 ) ) ;
#3696=CARTESIAN_POINT ( 'NONE',  ( 8.749999999999918288, 2.500000000000000000, 7.188010851410848723 ) ) ;
#3697=ORIENTED_EDGE ( 'NONE', *, *, #53423, .F. ) ;
#3698=ORIENTED_EDGE ( 'NONE', *, *, #124964, .T. ) ;
#3699=EDGE_LOOP ( 'NONE', ( #11441, #94975, #65024, #118324 ) ) ;
#3700=EDGE_LOOP ( 'NONE', ( #99315, #7947, #516, #125987 ) ) ;
#3701=ORIENTED_EDGE ( 'NONE', *, *, #2633, .F. ) ;
#3702=CARTESIAN_POINT ( 'NONE',  ( -4.350000000000023626, 2.500000000000000000, -2.411473670974877859 ) ) ;
#3703=CARTESIAN_POINT ( 'NONE',  ( -1.700000000000035261, 2.500000000000000000, 4.330127018922196314 ) ) ;
#3704=ORIENTED_EDGE ( 'NONE', *, *, #13493, .T. ) ;
#3705=ADVANCED_FACE ( 'NONE', ( #91533 ), #71236, .T. ) ;
#3706=FACE_BOUND ( 'NONE', #49713, .T. ) ;
#3707=CARTESIAN_POINT ( 'NONE',  ( -10.40000000000000213, 12.50000000000000000, 0.6928203230275494784 ) ) ;
#3708=CIRCLE ( 'NONE', #37084, 0.1000000000000002554 ) ;
#3709=CIRCLE ( 'NONE', #41386, 0.06509327318403745899 ) ;
#3710=EDGE_LOOP ( 'NONE', ( #1834, #128726 ) ) ;
#3711=FACE_OUTER_BOUND ( 'NONE', #44079, .T. ) ;
#3712=EDGE_CURVE ( 'NONE', #111704, #110043, #22812, .T. ) ;
#3713=CARTESIAN_POINT ( 'NONE',  ( 13.74999999999993427, 2.500000000000000000, 2.065063509461097624 ) ) ;
#3714=CARTESIAN_POINT ( 'NONE',  ( -3.150000000000029221, 12.50000000000000000, 2.511473670974873507 ) ) ;
#3715=ORIENTED_EDGE ( 'NONE', *, *, #67545, .F. ) ;
#3716=FACE_OUTER_BOUND ( 'NONE', #51286, .T. ) ;
#3717=CONICAL_SURFACE ( 'NONE', #127071, 0.09999999999999982514, 0.003490658503988666988 ) ;
#3719=CIRCLE ( 'NONE', #64358, 0.09999999999999982514 ) ;
#3720=AXIS2_PLACEMENT_3D ( 'NONE', #118679, #117360, #8078 ) ;
#3722=ORIENTED_EDGE ( 'NONE', *, *, #66414, .F. ) ;
#3723=LINE ( 'NONE', #33829, #25467 ) ;
#3724=FACE_OUTER_BOUND ( 'NONE', #67466, .T. ) ;
#3725=DIRECTION ( 'NONE',  ( 0.000000000000000000, 0.000000000000000000, -1.000000000000000000 ) ) ;
#3726=ORIENTED_EDGE ( 'NONE', *, *, #79808, .F. ) ;
#3727=CARTESIAN_POINT ( 'NONE',  ( 4.999999999999935163, 2.500000000000000000, 3.637306695894644726 ) ) ;
#3728=AXIS2_PLACEMENT_3D ( 'NONE', #121084, #90313, #32081 ) ;
#3729=LINE ( 'NONE', #73124, #94928 ) ;
#3730=ADVANCED_FACE ( 'NONE', ( #71904 ), #82373, .T. ) ;
#3731=DIRECTION ( 'NONE',  ( 0.000000000000000000, 0.000000000000000000, 1.000000000000000000 ) ) ;
#3733=ORIENTED_EDGE ( 'NONE', *, *, #54546, .F. ) ;
#3734=CONICAL_SURFACE ( 'NONE', #118655, 0.1000000000000000472, 0.003490658503988666988 ) ;
#3735=DIRECTION ( 'NONE',  ( 0.000000000000000000, 0.000000000000000000, 1.000000000000000000 ) ) ;
#3737=DIRECTION ( 'NONE',  ( 0.000000000000000000, 0.000000000000000000, 1.000000000000000000 ) ) ;
#3738=EDGE_CURVE ( 'NONE', #19521, #87479, #72551, .T. ) ;
#3739=AXIS2_PLACEMENT_3D ( 'NONE', #21719, #29598, #69513 ) ;
#3740=ORIENTED_EDGE ( 'NONE', *, *, #99667, .F. ) ;
#3741=VERTEX_POINT ( 'NONE', #15529 ) ;
#3742=CARTESIAN_POINT ( 'NONE',  ( 5.449999999999936229, 12.50000000000000000, -2.165063509461101710 ) ) ;
#3743=CIRCLE ( 'NONE', #28896, 0.09999999999999999167 ) ;
#3744=DIRECTION ( 'NONE',  ( -0.000000000000000000, 1.000000000000000000, -0.000000000000000000 ) ) ;
#3745=ADVANCED_FACE ( 'NONE', ( #104567 ), #51972, .T. ) ;
#3746=DIRECTION ( 'NONE',  ( 0.000000000000000000, -0.000000000000000000, 1.000000000000000000 ) ) ;
#3747=DIRECTION ( 'NONE',  ( -0.000000000000000000, 1.000000000000000000, -0.000000000000000000 ) ) ;
#3748=EDGE_CURVE ( 'NONE', #87862, #69423, #122934, .T. ) ;
#3751=AXIS2_PLACEMENT_3D ( 'NONE', #118047, #78143, #26462 ) ;
#3752=ADVANCED_FACE ( 'NONE', ( #45663 ), #103932, .T. ) ;
#3753=VERTEX_POINT ( 'NONE', #43105 ) ;
#3754=ORIENTED_EDGE ( 'NONE', *, *, #119805, .T. ) ;
#3755=CARTESIAN_POINT ( 'NONE',  ( -12.94999999999999218, 2.500000000000000000, 2.265063509461101354 ) ) ;
#3756=CIRCLE ( 'NONE', #16249, 0.09999999999999982514 ) ;
#3757=CARTESIAN_POINT ( 'NONE',  ( -14.14999999999998614, 2.500000000000000000, 1.372243186433549367 ) ) ;
#3758=EDGE_CURVE ( 'NONE', #8949, #106738, #56052, .T. ) ;
#3759=CARTESIAN_POINT ( 'NONE',  ( -12.09999999999999609, 12.50000000000000000, -4.957854068765714217 ) ) ;
#3760=ORIENTED_EDGE ( 'NONE', *, *, #90054, .F. ) ;
#3761=EDGE_LOOP ( 'NONE', ( #59190, #119473, #24482, #32735 ) ) ;
#3762=EDGE_CURVE ( 'NONE', #92740, #119776, #93726, .T. ) ;
#3763=DIRECTION ( 'NONE',  ( 0.000000000000000000, 0.000000000000000000, 1.000000000000000000 ) ) ;
#3764=AXIS2_PLACEMENT_3D ( 'NONE', #90489, #1469, #108842 ) ;
#3765=VERTEX_POINT ( 'NONE', #114380 ) ;
#3766=DIRECTION ( 'NONE',  ( 0.000000000000000000, 0.000000000000000000, 1.000000000000000000 ) ) ;
#3767=EDGE_CURVE ( 'NONE', #110204, #88926, #129260, .T. ) ;
#3768=CIRCLE ( 'NONE', #112447, 0.1000000000000000472 ) ;
#3769=ADVANCED_FACE ( 'NONE', ( #3794 ), #79166, .T. ) ;
#3770=CARTESIAN_POINT ( 'NONE',  ( -12.89999999999999147, 2.500000000000000000, 5.022947341949748790 ) ) ;
#3771=ORIENTED_EDGE ( 'NONE', *, *, #91696, .T. ) ;
#3772=DIRECTION ( 'NONE',  ( 0.000000000000000000, 0.000000000000000000, -1.000000000000000000 ) ) ;
#3773=DIRECTION ( 'NONE',  ( 0.000000000000000000, 0.000000000000000000, -1.000000000000000000 ) ) ;
#3774=DIRECTION ( 'NONE',  ( -0.000000000000000000, -1.000000000000000000, -0.000000000000000000 ) ) ;
#3775=CIRCLE ( 'NONE', #120754, 0.09999999999999982514 ) ;
#3776=ADVANCED_FACE ( 'NONE', ( #73813 ), #129350, .T. ) ;
#3777=DIRECTION ( 'NONE',  ( 0.000000000000000000, 0.000000000000000000, -1.000000000000000000 ) ) ;
#3778=EDGE_CURVE ( 'NONE', #77998, #16575, #75115, .T. ) ;
#3779=ORIENTED_EDGE ( 'NONE', *, *, #70904, .F. ) ;
#3780=LINE ( 'NONE', #52883, #15250 ) ;
#3781=CIRCLE ( 'NONE', #91605, 0.06509327318403741736 ) ;
#3782=AXIS2_PLACEMENT_3D ( 'NONE', #3353, #13148, #84495 ) ;
#3783=CARTESIAN_POINT ( 'NONE',  ( 87.50000000000001421, -3.974992050023846257, 6.359987280038161828 ) ) ;
#3784=ORIENTED_EDGE ( 'NONE', *, *, #101609, .F. ) ;
#3785=ORIENTED_EDGE ( 'NONE', *, *, #45553, .F. ) ;
#3787=DIRECTION ( 'NONE',  ( 0.000000000000000000, 0.000000000000000000, -1.000000000000000000 ) ) ;
#3788=DIRECTION ( 'NONE',  ( 0.000000000000000000, 0.000000000000000000, -1.000000000000000000 ) ) ;
#3789=DIRECTION ( 'NONE',  ( -0.000000000000000000, -1.000000000000000000, -0.000000000000000000 ) ) ;
#3790=LINE ( 'NONE', #52252, #2527 ) ;
#3791=DIRECTION ( 'NONE',  ( -4.274815082592931898E-19, -0.9999939076577903929, -0.003490651415223739937 ) ) ;
#3792=CARTESIAN_POINT ( 'NONE',  ( -0.6500000000000398792, 2.500000000000000000, -6.841600689897078702 ) ) ;
#3793=CARTESIAN_POINT ( 'NONE',  ( 5.449999999999934452, 2.500000000000000000, 2.165063509461097713 ) ) ;
#3794=FACE_OUTER_BOUND ( 'NONE', #102990, .T. ) ;
#3795=FACE_OUTER_BOUND ( 'NONE', #13437, .T. ) ;
#3796=DIRECTION ( 'NONE',  ( 0.000000000000000000, 1.000000000000000000, 0.000000000000000000 ) ) ;
#3797=ORIENTED_EDGE ( 'NONE', *, *, #63918, .F. ) ;
#3798=VERTEX_POINT ( 'NONE', #95397 ) ;
#3799=ORIENTED_EDGE ( 'NONE', *, *, #41172, .T. ) ;
#3800=AXIS2_PLACEMENT_3D ( 'NONE', #89704, #39971, #122400 ) ;
#3801=AXIS2_PLACEMENT_3D ( 'NONE', #92100, #3097, #50910 ) ;
#3802=ORIENTED_EDGE ( 'NONE', *, *, #74124, .F. ) ;
#3803=CARTESIAN_POINT ( 'NONE',  ( -13.74999999999998934, 12.50000000000000000, 2.857883832488652853 ) ) ;
#3804=DIRECTION ( 'NONE',  ( 0.000000000000000000, 0.000000000000000000, 1.000000000000000000 ) ) ;
#3805=EDGE_LOOP ( 'NONE', ( #88306, #97818 ) ) ;
#3806=AXIS2_PLACEMENT_3D ( 'NONE', #44021, #74125, #76049 ) ;
#3807=DIRECTION ( 'NONE',  ( 0.000000000000000000, 0.000000000000000000, -1.000000000000000000 ) ) ;
#3808=EDGE_CURVE ( 'NONE', #948, #47249, #39464, .T. ) ;
#3809=EDGE_CURVE ( 'NONE', #49723, #50793, #53548, .T. ) ;
#3810=DIRECTION ( 'NONE',  ( -0.000000000000000000, -1.000000000000000000, -0.000000000000000000 ) ) ;
#3811=PLANE ( 'NONE',  #51676 ) ;
#3812=ORIENTED_EDGE ( 'NONE', *, *, #27823, .T. ) ;
#3813=CARTESIAN_POINT ( 'NONE',  ( -9.400000000000009237, 12.50000000000000000, -4.048810130592459089 ) ) ;
#3814=AXIS2_PLACEMENT_3D ( 'NONE', #77719, #67233, #39773 ) ;
#3816=ORIENTED_EDGE ( 'NONE', *, *, #65092, .F. ) ;
#3817=CIRCLE ( 'NONE', #110424, 0.1000000000000002554 ) ;
#3818=ORIENTED_EDGE ( 'NONE', *, *, #108538, .T. ) ;
#3820=ORIENTED_EDGE ( 'NONE', *, *, #112260, .F. ) ;
#3821=DIRECTION ( 'NONE',  ( 0.000000000000000000, -0.9999939076577903929, 0.003490651415223739937 ) ) ;
#3822=DIRECTION ( 'NONE',  ( 0.000000000000000000, 0.000000000000000000, -1.000000000000000000 ) ) ;
#3823=DIRECTION ( 'NONE',  ( -4.274815082592931898E-19, -0.9999939076577903929, -0.003490651415223739937 ) ) ;
#3824=DIRECTION ( 'NONE',  ( 0.000000000000000000, 0.000000000000000000, 1.000000000000000000 ) ) ;
#3825=CIRCLE ( 'NONE', #16322, 0.09999999999999982514 ) ;
#3826=ORIENTED_EDGE ( 'NONE', *, *, #27112, .F. ) ;
#3827=CARTESIAN_POINT ( 'NONE',  ( 13.74999999999989342, 2.500000000000000000, -1.372243186433550033 ) ) ;
#3828=ORIENTED_EDGE ( 'NONE', *, *, #65772, .F. ) ;
#3831=CARTESIAN_POINT ( 'NONE',  ( -2.100000000000034284, 12.50000000000000000, -4.265033745738164406 ) ) ;
#3832=DIRECTION ( 'NONE',  ( 0.000000000000000000, 0.000000000000000000, 1.000000000000000000 ) ) ;
#3833=DIRECTION ( 'NONE',  ( 0.000000000000000000, 0.000000000000000000, -1.000000000000000000 ) ) ;
#3834=EDGE_LOOP ( 'NONE', ( #21102, #73586 ) ) ;
#3835=AXIS2_PLACEMENT_3D ( 'NONE', #110524, #30698, #20857 ) ;
#3836=ORIENTED_EDGE ( 'NONE', *, *, #495, .T. ) ;
#3838=DIRECTION ( 'NONE',  ( 0.000000000000000000, 0.000000000000000000, 1.000000000000000000 ) ) ;
#3839=DIRECTION ( 'NONE',  ( 0.000000000000000000, 1.000000000000000000, 0.000000000000000000 ) ) ;
#3840=CARTESIAN_POINT ( 'NONE',  ( 5.199999999999933564, 2.500000000000000000, 3.883716857408420431 ) ) ;
#3841=FACE_BOUND ( 'NONE', #38528, .T. ) ;
#3842=DIRECTION ( 'NONE',  ( -0.000000000000000000, 1.000000000000000000, -0.000000000000000000 ) ) ;
#3843=FACE_OUTER_BOUND ( 'NONE', #17918, .T. ) ;
#3845=DIRECTION ( 'NONE',  ( 0.000000000000000000, 1.000000000000000000, 0.000000000000000000 ) ) ;
#3846=EDGE_CURVE ( 'NONE', #89337, #99110, #33198, .T. ) ;
#3847=AXIS2_PLACEMENT_3D ( 'NONE', #81887, #102204, #61635 ) ;
#3848=PLANE ( 'NONE',  #86042 ) ;
#3849=DIRECTION ( 'NONE',  ( 0.000000000000000000, 0.000000000000000000, 1.000000000000000000 ) ) ;
#3850=CIRCLE ( 'NONE', #77014, 0.06509327318403745899 ) ;
#3851=DIRECTION ( 'NONE',  ( -0.000000000000000000, -1.000000000000000000, -0.000000000000000000 ) ) ;
#3852=EDGE_LOOP ( 'NONE', ( #13495, #15911 ) ) ;
#3853=FACE_OUTER_BOUND ( 'NONE', #7082, .T. ) ;
#3854=VERTEX_POINT ( 'NONE', #14241 ) ;
#3855=VERTEX_POINT ( 'NONE', #54192 ) ;
#3856=ORIENTED_EDGE ( 'NONE', *, *, #12301, .T. ) ;
#3857=ORIENTED_EDGE ( 'NONE', *, *, #115140, .T. ) ;
#3858=EDGE_CURVE ( 'NONE', #129477, #96927, #124932, .T. ) ;
#3859=CIRCLE ( 'NONE', #79093, 0.06509327318403745899 ) ;
#3860=CARTESIAN_POINT ( 'NONE',  ( 6.049999999999932321, 12.50000000000000000, 1.818653347947321475 ) ) ;
#3861=EDGE_CURVE ( 'NONE', #39180, #29091, #50734, .T. ) ;
#3862=FACE_BOUND ( 'NONE', #66098, .T. ) ;
#3863=CARTESIAN_POINT ( 'NONE',  ( -8.750000000000010658, 12.50000000000000000, -1.472243186433550122 ) ) ;
#3864=CIRCLE ( 'NONE', #6001, 0.1000000000000002554 ) ;
#3865=AXIS2_PLACEMENT_3D ( 'NONE', #54842, #113130, #3824 ) ;
#3866=EDGE_LOOP ( 'NONE', ( #80262, #68192, #74858, #27927 ) ) ;
#3867=CARTESIAN_POINT ( 'NONE',  ( -10.40000000000000213, 12.50000000000000000, 5.022947341949748790 ) ) ;
#3868=EDGE_CURVE ( 'NONE', #40568, #79650, #11451, .T. ) ;
#3869=DIRECTION ( 'NONE',  ( 0.000000000000000000, 1.000000000000000000, 0.000000000000000000 ) ) ;
#3870=ORIENTED_EDGE ( 'NONE', *, *, #80627, .T. ) ;
#3871=FACE_OUTER_BOUND ( 'NONE', #119901, .T. ) ;
#3872=DIRECTION ( 'NONE',  ( 0.000000000000000000, 0.000000000000000000, -1.000000000000000000 ) ) ;
#3873=EDGE_LOOP ( 'NONE', ( #36112, #11181, #64218, #103097 ) ) ;
#3874=VECTOR ( 'NONE', #31558, 1000.000000000000000 ) ;
#3875=CARTESIAN_POINT ( 'NONE',  ( -13.74999999999998757, 2.500000000000000000, 1.472243186433549456 ) ) ;
#3876=CARTESIAN_POINT ( 'NONE',  ( 8.549999999999924327, 12.50000000000000000, 1.883746621131358934 ) ) ;
#3877=ORIENTED_EDGE ( 'NONE', *, *, #112479, .F. ) ;
#3878=CIRCLE ( 'NONE', #62396, 0.1000000000000000472 ) ;
#3879=FACE_OUTER_BOUND ( 'NONE', #50222, .T. ) ;
#3882=AXIS2_PLACEMENT_3D ( 'NONE', #124833, #73784, #33860 ) ;
#3883=DIRECTION ( 'NONE',  ( 0.000000000000000000, -0.9999939076577903929, 0.003490651415223739937 ) ) ;
#3884=ORIENTED_EDGE ( 'NONE', *, *, #43676, .T. ) ;
#3885=EDGE_LOOP ( 'NONE', ( #5495, #46002 ) ) ;
#3886=FACE_OUTER_BOUND ( 'NONE', #124097, .T. ) ;
#3887=AXIS2_PLACEMENT_3D ( 'NONE', #58649, #77618, #67808 ) ;
#3888=ORIENTED_EDGE ( 'NONE', *, *, #106009, .T. ) ;
#3889=PLANE ( 'NONE',  #42915 ) ;
#3890=CARTESIAN_POINT ( 'NONE',  ( 10.79999999999991367, 12.50000000000000000, -2.385244779468109755E-15 ) ) ;
#3891=EDGE_CURVE ( 'NONE', #108508, #7948, #21937, .T. ) ;
#3892=VERTEX_POINT ( 'NONE', #110299 ) ;
#3893=CIRCLE ( 'NONE', #100055, 0.1000000000000000472 ) ;
#3894=CARTESIAN_POINT ( 'NONE',  ( 0.8499999999999536815, 2.500000000000000000, 6.395190528383296602 ) ) ;
#3895=CARTESIAN_POINT ( 'NONE',  ( 6.899999999999928413, 12.50000000000000000, 4.741630453620009789 ) ) ;
#3896=CARTESIAN_POINT ( 'NONE',  ( -3.350000000000029399, 12.50000000000000000, 6.495190528383297135 ) ) ;
#3897=LINE ( 'NONE', #14979, #96754 ) ;
#3898=ADVANCED_FACE ( 'NONE', ( #81490 ), #101127, .T. ) ;
#3899=DIRECTION ( 'NONE',  ( -0.000000000000000000, -1.000000000000000000, -0.000000000000000000 ) ) ;
#3900=CONICAL_SURFACE ( 'NONE', #77068, 0.1000000000000002554, 0.003490658503988666988 ) ;
#3901=EDGE_CURVE ( 'NONE', #18217, #5550, #32418, .T. ) ;
#3902=VERTEX_POINT ( 'NONE', #43514 ) ;
#3903=VECTOR ( 'NONE', #107310, 1000.000000000000000 ) ;
#3904=ORIENTED_EDGE ( 'NONE', *, *, #36602, .F. ) ;
#3905=DIRECTION ( 'NONE',  ( -0.000000000000000000, -1.000000000000000000, -0.000000000000000000 ) ) ;
#3906=CARTESIAN_POINT ( 'NONE',  ( -8.950000000000009948, 2.500000000000000000, -6.941600689897073018 ) ) ;
#3907=ADVANCED_FACE ( 'NONE', ( #22592 ), #3566, .T. ) ;
#3908=ORIENTED_EDGE ( 'NONE', *, *, #129083, .F. ) ;
#3909=ORIENTED_EDGE ( 'NONE', *, *, #54295, .F. ) ;
#3910=EDGE_CURVE ( 'NONE', #14174, #79060, #82793, .T. ) ;
#3911=ORIENTED_EDGE ( 'NONE', *, *, #25247, .F. ) ;
#3912=ADVANCED_FACE ( 'NONE', ( #2260 ), #89336, .T. ) ;
#3913=FACE_OUTER_BOUND ( 'NONE', #29405, .T. ) ;
#3914=CARTESIAN_POINT ( 'NONE',  ( 5.649999999999932854, 2.500000000000000000, 2.511473670974873507 ) ) ;
#3917=EDGE_CURVE ( 'NONE', #101225, #114688, #108197, .T. ) ;
#3918=CARTESIAN_POINT ( 'NONE',  ( -6.250000000000017764, 12.50000000000000000, 7.122917578226811486 ) ) ;
#3919=CARTESIAN_POINT ( 'NONE',  ( 6.899999999999928413, 2.500000000000000000, 4.676537180435972552 ) ) ;
#3920=DIRECTION ( 'NONE',  ( -4.274815082592931898E-19, -0.9999939076577903929, -0.003490651415223739937 ) ) ;
#3921=DIRECTION ( 'NONE',  ( 0.000000000000000000, 0.000000000000000000, 1.000000000000000000 ) ) ;
#3922=AXIS2_PLACEMENT_3D ( 'NONE', #51784, #9919, #19753 ) ;
#3923=DIRECTION ( 'NONE',  ( 0.000000000000000000, 0.000000000000000000, 1.000000000000000000 ) ) ;
#3924=DIRECTION ( 'NONE',  ( -0.000000000000000000, 1.000000000000000000, -0.000000000000000000 ) ) ;
#3925=ADVANCED_FACE ( 'NONE', ( #112238 ), #26642, .T. ) ;
#3926=EDGE_LOOP ( 'NONE', ( #49968, #127080 ) ) ;
#3927=LINE ( 'NONE', #123070, #48573 ) ;
#3928=ORIENTED_EDGE ( 'NONE', *, *, #21995, .F. ) ;
#3929=ORIENTED_EDGE ( 'NONE', *, *, #57386, .T. ) ;
#3930=CARTESIAN_POINT ( 'NONE',  ( -9.150000000000009237, 2.500000000000000000, 1.472243186433545459 ) ) ;
#3931=DIRECTION ( 'NONE',  ( -0.000000000000000000, -1.000000000000000000, -0.000000000000000000 ) ) ;
#3932=CIRCLE ( 'NONE', #98022, 0.1000000000000002554 ) ;
#3933=DIRECTION ( 'NONE',  ( 0.000000000000000000, 0.000000000000000000, 1.000000000000000000 ) ) ;
#3934=FACE_OUTER_BOUND ( 'NONE', #103769, .T. ) ;
#3935=AXIS2_PLACEMENT_3D ( 'NONE', #84489, #85759, #54372 ) ;
#3936=DIRECTION ( 'NONE',  ( -4.274815082592931898E-19, -0.9999939076577903929, -0.003490651415223739937 ) ) ;
#3937=DIRECTION ( 'NONE',  ( 0.000000000000000000, 0.000000000000000000, 1.000000000000000000 ) ) ;
#3938=DIRECTION ( 'NONE',  ( 0.000000000000000000, -0.000000000000000000, 1.000000000000000000 ) ) ;
#3939=VERTEX_POINT ( 'NONE', #82129 ) ;
#3940=DIRECTION ( 'NONE',  ( 0.000000000000000000, -1.000000000000000000, 0.000000000000000000 ) ) ;
#3941=CIRCLE ( 'NONE', #108491, 0.06509327318403745899 ) ;
#3942=LINE ( 'NONE', #43892, #106478 ) ;
#3943=VERTEX_POINT ( 'NONE', #100476 ) ;
#3944=ORIENTED_EDGE ( 'NONE', *, *, #101444, .F. ) ;
#3945=AXIS2_PLACEMENT_3D ( 'NONE', #72081, #86212, #111317 ) ;
#3946=CIRCLE ( 'NONE', #81322, 0.06509327318403745899 ) ;
#3947=EDGE_LOOP ( 'NONE', ( #28074, #39248 ) ) ;
#3948=AXIS2_PLACEMENT_3D ( 'NONE', #90804, #60077, #1134 ) ;
#3949=ORIENTED_EDGE ( 'NONE', *, *, #129074, .T. ) ;
#3950=LINE ( 'NONE', #14405, #21060 ) ;
#3951=CARTESIAN_POINT ( 'NONE',  ( 4.599999999999940137, 2.500000000000000000, -4.330127018922201643 ) ) ;
#3952=CIRCLE ( 'NONE', #54137, 0.09999999999999982514 ) ;
#3953=CIRCLE ( 'NONE', #66643, 0.06509327318403745899 ) ;
#3954=CARTESIAN_POINT ( 'NONE',  ( -1.650000000000034328, 2.500000000000000000, -6.595190528383302109 ) ) ;
#3955=EDGE_CURVE ( 'NONE', #112224, #100139, #74765, .T. ) ;
#3956=CARTESIAN_POINT ( 'NONE',  ( 4.549999999999937650, 2.500000000000000000, 2.165063509461097713 ) ) ;
#3957=DIRECTION ( 'NONE',  ( 0.000000000000000000, 0.000000000000000000, 1.000000000000000000 ) ) ;
#3958=ORIENTED_EDGE ( 'NONE', *, *, #53560, .F. ) ;
#3959=DIRECTION ( 'NONE',  ( 0.000000000000000000, -0.000000000000000000, 1.000000000000000000 ) ) ;
#3960=DIRECTION ( 'NONE',  ( 0.000000000000000000, 1.000000000000000000, 0.000000000000000000 ) ) ;
#3961=CARTESIAN_POINT ( 'NONE',  ( -2.300000000000033129, 2.500000000000000000, 3.883716857408420431 ) ) ;
#3963=EDGE_CURVE ( 'NONE', #13704, #125289, #12093, .T. ) ;
#3964=ORIENTED_EDGE ( 'NONE', *, *, #9519, .T. ) ;
#3965=VERTEX_POINT ( 'NONE', #12723 ) ;
#3966=ORIENTED_EDGE ( 'NONE', *, *, #49932, .T. ) ;
#3967=CIRCLE ( 'NONE', #56190, 0.06509327318403745899 ) ;
#3968=CARTESIAN_POINT ( 'NONE',  ( -13.34999999999999076, 2.500000000000000000, 1.472243186433549456 ) ) ;
#3969=CARTESIAN_POINT ( 'NONE',  ( 4.799999999999935874, 2.500000000000000000, 3.883716857408421319 ) ) ;
#3970=CARTESIAN_POINT ( 'NONE',  ( 13.54999999999990123, 12.50000000000000000, 1.753560074763284016 ) ) ;
#3971=CONICAL_SURFACE ( 'NONE', #85448, 0.1000000000000000472, 0.003490658503988666988 ) ;
#3972=AXIS2_PLACEMENT_3D ( 'NONE', #22173, #119691, #31983 ) ;
#3973=ORIENTED_EDGE ( 'NONE', *, *, #3234, .T. ) ;
#3974=FACE_OUTER_BOUND ( 'NONE', #25334, .T. ) ;
#3975=DIRECTION ( 'NONE',  ( -0.000000000000000000, 1.000000000000000000, -0.000000000000000000 ) ) ;
#3976=CARTESIAN_POINT ( 'NONE',  ( 5.649999999999934630, 12.50000000000000000, -2.446380397790840266 ) ) ;
#3977=CARTESIAN_POINT ( 'NONE',  ( -9.999999999999969802, 12.50000000000000000, -0.06509327318403970719 ) ) ;
#3978=CARTESIAN_POINT ( 'NONE',  ( 0.000000000000000000, 12.50000000000000000, 0.000000000000000000 ) ) ;
#3979=ORIENTED_EDGE ( 'NONE', *, *, #107477, .T. ) ;
#3980=ORIENTED_EDGE ( 'NONE', *, *, #112367, .T. ) ;
#3981=DIRECTION ( 'NONE',  ( 0.000000000000000000, -0.9999939076577903929, 0.003490651415223739937 ) ) ;
#3982=PLANE ( 'NONE',  #123004 ) ;
#3983=CIRCLE ( 'NONE', #8191, 0.09999999999999982514 ) ;
#3984=DIRECTION ( 'NONE',  ( -0.000000000000000000, 1.000000000000000000, -0.000000000000000000 ) ) ;
#3985=CARTESIAN_POINT ( 'NONE',  ( -12.94999999999999218, 2.500000000000000000, -2.165063509461099489 ) ) ;
#3986=DIRECTION ( 'NONE',  ( -0.000000000000000000, 1.000000000000000000, -0.000000000000000000 ) ) ;
#3987=CIRCLE ( 'NONE', #66686, 0.1000000000000002554 ) ;
#3988=EDGE_CURVE ( 'NONE', #17860, #112869, #52036, .T. ) ;
#3989=ORIENTED_EDGE ( 'NONE', *, *, #102534, .F. ) ;
#3990=ORIENTED_EDGE ( 'NONE', *, *, #102157, .T. ) ;
#3992=ADVANCED_FACE ( 'NONE', ( #52663 ), #92595, .T. ) ;
#3993=CARTESIAN_POINT ( 'NONE',  ( -1.450000000000035927, 12.50000000000000000, -6.148780366869526226 ) ) ;
#3994=CARTESIAN_POINT ( 'NONE',  ( 16.56576425165007294, -2.500000000000000000, -6.084390597445819893 ) ) ;
#3995=DIRECTION ( 'NONE',  ( -0.000000000000000000, 1.000000000000000000, -0.000000000000000000 ) ) ;
#3996=ORIENTED_EDGE ( 'NONE', *, *, #58573, .F. ) ;
#3997=EDGE_CURVE ( 'NONE', #70661, #49409, #28796, .T. ) ;
#3998=DIRECTION ( 'NONE',  ( 0.000000000000000000, 1.000000000000000000, 0.000000000000000000 ) ) ;
#3999=DIRECTION ( 'NONE',  ( 0.000000000000000000, 0.000000000000000000, 1.000000000000000000 ) ) ;
#4000=VECTOR ( 'NONE', #10247, 1000.000000000000000 ) ;
#4001=ORIENTED_EDGE ( 'NONE', *, *, #123718, .T. ) ;
#4002=EDGE_CURVE ( 'NONE', #54614, #97758, #112884, .T. ) ;
#4003=CARTESIAN_POINT ( 'NONE',  ( 8.099999999999923261, 2.500000000000000000, 3.983716857408420076 ) ) ;
#4004=EDGE_CURVE ( 'NONE', #26833, #81036, #85220, .T. ) ;
#4005=ORIENTED_EDGE ( 'NONE', *, *, #110608, .T. ) ;
#4006=CARTESIAN_POINT ( 'NONE',  ( -12.69999999999999218, 12.50000000000000000, -4.676537180435975216 ) ) ;
#4007=ORIENTED_EDGE ( 'NONE', *, *, #99264, .F. ) ;
#4008=CARTESIAN_POINT ( 'NONE',  ( 4.149999999999938183, 12.50000000000000000, 2.099970236277060032 ) ) ;
#4009=DIRECTION ( 'NONE',  ( 0.000000000000000000, 1.000000000000000000, 0.000000000000000000 ) ) ;
#4010=EDGE_CURVE ( 'NONE', #49054, #40465, #60395, .T. ) ;
#4011=ORIENTED_EDGE ( 'NONE', *, *, #52884, .F. ) ;
#4012=ORIENTED_EDGE ( 'NONE', *, *, #66461, .T. ) ;
#4013=ADVANCED_FACE ( 'NONE', ( #113515 ), #126991, .T. ) ;
#4015=CARTESIAN_POINT ( 'NONE',  ( 14.59999999999989484, 2.500000000000000000, -2.276824562219559311E-15 ) ) ;
#4016=VECTOR ( 'NONE', #879, 1000.000000000000000 ) ;
#4017=DIRECTION ( 'NONE',  ( 0.000000000000000000, 1.000000000000000000, 0.000000000000000000 ) ) ;
#4019=CARTESIAN_POINT ( 'NONE',  ( 8.749999999999918288, 12.50000000000000000, -1.407149913249512663 ) ) ;
#4020=DIRECTION ( 'NONE',  ( 0.000000000000000000, 1.000000000000000000, 0.000000000000000000 ) ) ;
#4021=DIRECTION ( 'NONE',  ( 0.000000000000000000, 0.000000000000000000, 1.000000000000000000 ) ) ;
#4022=CARTESIAN_POINT ( 'NONE',  ( -1.050000000000038236, 2.500000000000000000, -1.718653347947326049 ) ) ;
#4023=AXIS2_PLACEMENT_3D ( 'NONE', #81368, #71521, #10037 ) ;
#4024=VERTEX_POINT ( 'NONE', #16587 ) ;
#4025=EDGE_LOOP ( 'NONE', ( #2773, #92321, #102969, #50377 ) ) ;
#4026=DIRECTION ( 'NONE',  ( 0.000000000000000000, 0.000000000000000000, 1.000000000000000000 ) ) ;
#4027=CIRCLE ( 'NONE', #54225, 0.1000000000000000472 ) ;
#4028=ORIENTED_EDGE ( 'NONE', *, *, #106933, .T. ) ;
#4029=CARTESIAN_POINT ( 'NONE',  ( -2.300000000000032685, 12.50000000000000000, -0.2813168883297409439 ) ) ;
#4030=DIRECTION ( 'NONE',  ( 0.000000000000000000, 0.000000000000000000, 1.000000000000000000 ) ) ;
#4031=CARTESIAN_POINT ( 'NONE',  ( -1.450000000000035039, 12.50000000000000000, -6.841600689897077814 ) ) ;
#4032=CIRCLE ( 'NONE', #58357, 0.1000000000000002554 ) ;
#4033=ORIENTED_EDGE ( 'NONE', *, *, #125096, .F. ) ;
#4034=ORIENTED_EDGE ( 'NONE', *, *, #25162, .F. ) ;
#4035=FACE_BOUND ( 'NONE', #85849, .T. ) ;
#4036=ORIENTED_EDGE ( 'NONE', *, *, #102433, .F. ) ;
#4037=CARTESIAN_POINT ( 'NONE',  ( 6.699999999999928235, 2.500000000000000000, -2.276824562219559311E-15 ) ) ;
#4039=ORIENTED_EDGE ( 'NONE', *, *, #91263, .T. ) ;
#4040=CARTESIAN_POINT ( 'NONE',  ( 3.149999999999944400, 2.500000000000000000, 1.918653347947321564 ) ) ;
#4041=AXIS2_PLACEMENT_3D ( 'NONE', #26014, #73175, #85564 ) ;
#4042=AXIS2_PLACEMENT_3D ( 'NONE', #120863, #71118, #118933 ) ;
#4043=DIRECTION ( 'NONE',  ( 0.000000000000000000, 0.000000000000000000, -1.000000000000000000 ) ) ;
#4044=EDGE_CURVE ( 'NONE', #62105, #10563, #70544, .T. ) ;
#4045=DIRECTION ( 'NONE',  ( 0.000000000000000000, -0.000000000000000000, 1.000000000000000000 ) ) ;
#4046=DIRECTION ( 'NONE',  ( 0.000000000000000000, 1.000000000000000000, 0.000000000000000000 ) ) ;
#4047=CARTESIAN_POINT ( 'NONE',  ( -9.150000000000005684, 12.50000000000000000, 7.188010851410848723 ) ) ;
#4048=FACE_OUTER_BOUND ( 'NONE', #73324, .T. ) ;
#4050=CARTESIAN_POINT ( 'NONE',  ( -7.900000000000014566, 2.500000000000000000, -5.022947341949754119 ) ) ;
#4051=DIRECTION ( 'NONE',  ( 0.000000000000000000, 1.000000000000000000, 0.000000000000000000 ) ) ;
#4052=ADVANCED_FACE ( 'NONE', ( #14013 ), #26927, .T. ) ;
#4053=ORIENTED_EDGE ( 'NONE', *, *, #111507, .T. ) ;
#4054=ORIENTED_EDGE ( 'NONE', *, *, #59311, .F. ) ;
#4055=VERTEX_POINT ( 'NONE', #44136 ) ;
#4056=DIRECTION ( 'NONE',  ( 0.000000000000000000, 1.000000000000000000, 0.000000000000000000 ) ) ;
#4057=ORIENTED_EDGE ( 'NONE', *, *, #38524, .T. ) ;
#4058=EDGE_CURVE ( 'NONE', #14402, #40007, #122785, .T. ) ;
#4059=ORIENTED_EDGE ( 'NONE', *, *, #105278, .F. ) ;
#4060=VERTEX_POINT ( 'NONE', #5481 ) ;
#4061=ORIENTED_EDGE ( 'NONE', *, *, #128557, .T. ) ;
#4062=EDGE_CURVE ( 'NONE', #75765, #89533, #37117, .T. ) ;
#4063=CARTESIAN_POINT ( 'NONE',  ( 8.349999999999919709, 2.500000000000000000, 7.188010851410848723 ) ) ;
#4064=EDGE_CURVE ( 'NONE', #95559, #31928, #64417, .T. ) ;
#4065=CIRCLE ( 'NONE', #129584, 0.1000000000000002554 ) ;
#4066=CONICAL_SURFACE ( 'NONE', #8266, 0.1000000000000000472, 0.003490658503988666988 ) ;
#4067=CARTESIAN_POINT ( 'NONE',  ( 4.349999999999941025, 12.50000000000000000, -1.818653347947326138 ) ) ;
#4068=ADVANCED_FACE ( 'NONE', ( #114800 ), #18310, .T. ) ;
#4069=CARTESIAN_POINT ( 'NONE',  ( 76.44836599025838098, -3.583082431487559560, -6.086789564813110509 ) ) ;
#4070=DIRECTION ( 'NONE',  ( 0.000000000000000000, -0.000000000000000000, 1.000000000000000000 ) ) ;
#4071=FACE_OUTER_BOUND ( 'NONE', #75868, .T. ) ;
#4072=ORIENTED_EDGE ( 'NONE', *, *, #56547, .F. ) ;
#4073=AXIS2_PLACEMENT_3D ( 'NONE', #33259, #64622, #84909 ) ;
#4074=LINE ( 'NONE', #23735, #18374 ) ;
#4075=EDGE_CURVE ( 'NONE', #79185, #78982, #85349, .T. ) ;
#4076=ORIENTED_EDGE ( 'NONE', *, *, #124165, .T. ) ;
#4077=CIRCLE ( 'NONE', #125075, 0.1000000000000002554 ) ;
#4078=ADVANCED_FACE ( 'NONE', ( #35615 ), #95596, .T. ) ;
#4079=ORIENTED_EDGE ( 'NONE', *, *, #21227, .T. ) ;
#4080=ORIENTED_EDGE ( 'NONE', *, *, #78238, .F. ) ;
#4081=CARTESIAN_POINT ( 'NONE',  ( 11.84999999999990372, 2.500000000000000000, -6.841600689897078702 ) ) ;
#4082=ORIENTED_EDGE ( 'NONE', *, *, #63387, .T. ) ;
#4083=ORIENTED_EDGE ( 'NONE', *, *, #120492, .F. ) ;
#4084=ORIENTED_EDGE ( 'NONE', *, *, #34946, .F. ) ;
#4085=CIRCLE ( 'NONE', #20821, 0.1000000000000002554 ) ;
#4086=CIRCLE ( 'NONE', #98174, 0.1000000000000002554 ) ;
#4087=CARTESIAN_POINT ( 'NONE',  ( 13.74999999999989342, 12.50000000000000000, -1.472243186433550122 ) ) ;
#4088=PLANE ( 'NONE',  #87641 ) ;
#4089=FACE_OUTER_BOUND ( 'NONE', #29347, .T. ) ;
#4090=DIRECTION ( 'NONE',  ( -0.000000000000000000, 1.000000000000000000, -0.000000000000000000 ) ) ;
#4091=CARTESIAN_POINT ( 'NONE',  ( -3.100000000000028511, 2.500000000000000000, -4.083716857408426826 ) ) ;
#4092=CARTESIAN_POINT ( 'NONE',  ( 10.39999999999991509, 2.500000000000000000, -0.7928203230275543412 ) ) ;
#4093=ORIENTED_EDGE ( 'NONE', *, *, #92540, .T. ) ;
#4094=CARTESIAN_POINT ( 'NONE',  ( 10.79999999999991012, 2.500000000000000000, 4.230127018922196669 ) ) ;
#4095=ORIENTED_EDGE ( 'NONE', *, *, #99675, .T. ) ;
#4096=DIRECTION ( 'NONE',  ( -0.000000000000000000, -1.000000000000000000, -0.000000000000000000 ) ) ;
#4098=EDGE_LOOP ( 'NONE', ( #47396, #72839 ) ) ;
#4099=ORIENTED_EDGE ( 'NONE', *, *, #122595, .T. ) ;
#4100=DIRECTION ( 'NONE',  ( 0.000000000000000000, 0.000000000000000000, 1.000000000000000000 ) ) ;
#4101=PLANE ( 'NONE',  #86081 ) ;
#4102=DIRECTION ( 'NONE',  ( 0.000000000000000000, -0.000000000000000000, 1.000000000000000000 ) ) ;
#4103=VERTEX_POINT ( 'NONE', #4835 ) ;
#4104=ORIENTED_EDGE ( 'NONE', *, *, #25081, .T. ) ;
#4105=DIRECTION ( 'NONE',  ( 0.000000000000000000, 0.000000000000000000, 1.000000000000000000 ) ) ;
#4106=CARTESIAN_POINT ( 'NONE',  ( -10.40000000000000213, 2.500000000000000000, -0.7928203230275542301 ) ) ;
#4107=FACE_OUTER_BOUND ( 'NONE', #44945, .T. ) ;
#4108=CARTESIAN_POINT ( 'NONE',  ( 12.09999999999990195, 12.50000000000000000, -0.06509327318403970719 ) ) ;
#4109=DIRECTION ( 'NONE',  ( 0.000000000000000000, 0.000000000000000000, 1.000000000000000000 ) ) ;
#4110=ADVANCED_FACE ( 'NONE', ( #65705 ), #54581, .T. ) ;
#4112=AXIS2_PLACEMENT_3D ( 'NONE', #119029, #29370, #67979 ) ;
#4113=ORIENTED_EDGE ( 'NONE', *, *, #98594, .F. ) ;
#4114=CARTESIAN_POINT ( 'NONE',  ( 9.149999999999916866, 12.50000000000000000, 5.802370205355744659 ) ) ;
#4115=DIRECTION ( 'NONE',  ( -0.000000000000000000, 1.000000000000000000, -0.000000000000000000 ) ) ;
#4116=AXIS2_PLACEMENT_3D ( 'NONE', #115513, #15379, #53404 ) ;
#4117=CIRCLE ( 'NONE', #58535, 0.06509327318403745899 ) ;
#4118=CONICAL_SURFACE ( 'NONE', #77292, 0.1000000000000000056, 0.003490658503988666988 ) ;
#4121=DIRECTION ( 'NONE',  ( 0.000000000000000000, 1.000000000000000000, 0.000000000000000000 ) ) ;
#4122=FACE_OUTER_BOUND ( 'NONE', #118413, .T. ) ;
#4123=DIRECTION ( 'NONE',  ( 0.000000000000000000, 0.000000000000000000, 1.000000000000000000 ) ) ;
#4124=VERTEX_POINT ( 'NONE', #105643 ) ;
#4125=AXIS2_PLACEMENT_3D ( 'NONE', #108901, #88638, #109573 ) ;
#4126=CIRCLE ( 'NONE', #6186, 0.06509327318403745899 ) ;
#4127=DIRECTION ( 'NONE',  ( -0.000000000000000000, -1.000000000000000000, -0.000000000000000000 ) ) ;
#4128=DIRECTION ( 'NONE',  ( -0.000000000000000000, 1.000000000000000000, -0.000000000000000000 ) ) ;
#4129=CARTESIAN_POINT ( 'NONE',  ( 5.849999999999933920, 12.50000000000000000, -2.099970236277064473 ) ) ;
#4130=VERTEX_POINT ( 'NONE', #55881 ) ;
#4131=CARTESIAN_POINT ( 'NONE',  ( -10.40000000000000213, 2.500000000000000000, 4.330127018922196314 ) ) ;
#4132=EDGE_LOOP ( 'NONE', ( #107418, #65072 ) ) ;
#4133=FACE_OUTER_BOUND ( 'NONE', #85494, .T. ) ;
#4134=VERTEX_POINT ( 'NONE', #6130 ) ;
#4135=LINE ( 'NONE', #55203, #110696 ) ;
#4136=CARTESIAN_POINT ( 'NONE',  ( -2.950000000000029932, 12.50000000000000000, -2.165063509461101710 ) ) ;
#4137=LINE ( 'NONE', #93199, #27645 ) ;
#4138=ORIENTED_EDGE ( 'NONE', *, *, #105334, .F. ) ;
#4139=AXIS2_PLACEMENT_3D ( 'NONE', #103644, #4765, #93187 ) ;
#4140=ADVANCED_FACE ( 'NONE', ( #33677 ), #93539, .T. ) ;
#4141=DIRECTION ( 'NONE',  ( 0.000000000000000000, 0.000000000000000000, -1.000000000000000000 ) ) ;
#4142=CIRCLE ( 'NONE', #108714, 0.06509327318403745899 ) ;
#4143=DIRECTION ( 'NONE',  ( 0.000000000000000000, 1.000000000000000000, 0.000000000000000000 ) ) ;
#4144=EDGE_CURVE ( 'NONE', #33469, #22448, #49642, .T. ) ;
#4145=ADVANCED_FACE ( 'NONE', ( #76181 ), #76820, .T. ) ;
#4147=CIRCLE ( 'NONE', #18748, 0.09999999999999999167 ) ;
#4148=DIRECTION ( 'NONE',  ( -4.274815082592931898E-19, -0.9999939076577903929, -0.003490651415223739937 ) ) ;
#4149=ORIENTED_EDGE ( 'NONE', *, *, #6410, .T. ) ;
#4150=VERTEX_POINT ( 'NONE', #53962 ) ;
#4151=CARTESIAN_POINT ( 'NONE',  ( 7.949999999999925571, 2.500000000000000000, -6.495190528383302464 ) ) ;
#4152=FACE_OUTER_BOUND ( 'NONE', #108400, .T. ) ;
#4153=ADVANCED_FACE ( 'NONE', ( #93888 ), #123973, .T. ) ;
#4154=ADVANCED_FACE ( 'NONE', ( #90430 ), #40072, .T. ) ;
#4155=CARTESIAN_POINT ( 'NONE',  ( -9.550000000000007816, 2.500000000000000000, -6.495190528383297135 ) ) ;
#4156=EDGE_CURVE ( 'NONE', #73914, #2455, #79986, .T. ) ;
#4157=EDGE_LOOP ( 'NONE', ( #44282, #80842 ) ) ;
#4158=EDGE_CURVE ( 'NONE', #28402, #33970, #24580, .T. ) ;
#4159=DIRECTION ( 'NONE',  ( 0.000000000000000000, 0.000000000000000000, 1.000000000000000000 ) ) ;
#4160=DIRECTION ( 'NONE',  ( 0.000000000000000000, 1.000000000000000000, 0.000000000000000000 ) ) ;
#4161=EDGE_LOOP ( 'NONE', ( #113793, #119172 ) ) ;
#4162=VECTOR ( 'NONE', #127772, 1000.000000000000000 ) ;
#4163=FACE_OUTER_BOUND ( 'NONE', #57142, .T. ) ;
#4164=DIRECTION ( 'NONE',  ( -0.000000000000000000, -1.000000000000000000, -0.000000000000000000 ) ) ;
#4165=CIRCLE ( 'NONE', #94074, 0.1000000000000000472 ) ;
#4166=CARTESIAN_POINT ( 'NONE',  ( -2.950000000000030376, 2.500000000000000000, 6.595190528383296780 ) ) ;
#4167=DIRECTION ( 'NONE',  ( 0.000000000000000000, 0.000000000000000000, 1.000000000000000000 ) ) ;
#4168=CARTESIAN_POINT ( 'NONE',  ( 9.149999999999916866, 12.50000000000000000, -1.472243186433550122 ) ) ;
#4169=AXIS2_PLACEMENT_3D ( 'NONE', #78619, #38026, #117198 ) ;
#4170=PLANE ( 'NONE',  #24238 ) ;
#4171=DIRECTION ( 'NONE',  ( -0.000000000000000000, 1.000000000000000000, -0.000000000000000000 ) ) ;
#4173=ORIENTED_EDGE ( 'NONE', *, *, #38049, .T. ) ;
#4174=EDGE_LOOP ( 'NONE', ( #84363, #39397, #101141, #45765 ) ) ;
#4175=EDGE_LOOP ( 'NONE', ( #125051, #72045 ) ) ;
#4177=AXIS2_PLACEMENT_3D ( 'NONE', #96245, #74046, #44589 ) ;
#4178=DIRECTION ( 'NONE',  ( 0.000000000000000000, 0.000000000000000000, 1.000000000000000000 ) ) ;
#4179=CARTESIAN_POINT ( 'NONE',  ( -10.45000000000000462, 12.50000000000000000, -2.165063509461097713 ) ) ;
#4180=LINE ( 'NONE', #36894, #55201 ) ;
#4181=ORIENTED_EDGE ( 'NONE', *, *, #61194, .T. ) ;
#4182=FACE_BOUND ( 'NONE', #25201, .T. ) ;
#4183=CARTESIAN_POINT ( 'NONE',  ( 4.999999999999936939, 12.50000000000000000, -0.6928203230275541413 ) ) ;
#4184=DIRECTION ( 'NONE',  ( -0.000000000000000000, -1.000000000000000000, -0.000000000000000000 ) ) ;
#4185=DIRECTION ( 'NONE',  ( -0.000000000000000000, 1.000000000000000000, -0.000000000000000000 ) ) ;
#4186=DIRECTION ( 'NONE',  ( 0.000000000000000000, 1.000000000000000000, 0.000000000000000000 ) ) ;
#4187=DIRECTION ( 'NONE',  ( 0.000000000000000000, 0.000000000000000000, -1.000000000000000000 ) ) ;
#4188=FACE_OUTER_BOUND ( 'NONE', #71687, .T. ) ;
#4189=DIRECTION ( 'NONE',  ( 0.000000000000000000, 0.000000000000000000, 1.000000000000000000 ) ) ;
#4190=DIRECTION ( 'NONE',  ( 0.000000000000000000, 1.000000000000000000, 0.000000000000000000 ) ) ;
#4191=EDGE_CURVE ( 'NONE', #67661, #66137, #774, .T. ) ;
#4192=CARTESIAN_POINT ( 'NONE',  ( -8.350000000000013856, 12.50000000000000000, -7.188010851410848723 ) ) ;
#4193=DIRECTION ( 'NONE',  ( 0.000000000000000000, 0.000000000000000000, -1.000000000000000000 ) ) ;
#4194=ORIENTED_EDGE ( 'NONE', *, *, #91505, .F. ) ;
#4195=ORIENTED_EDGE ( 'NONE', *, *, #62156, .T. ) ;
#4196=ORIENTED_EDGE ( 'NONE', *, *, #18388, .T. ) ;
#4197=ORIENTED_EDGE ( 'NONE', *, *, #40606, .T. ) ;
#4198=VERTEX_POINT ( 'NONE', #32203 ) ;
#4199=EDGE_LOOP ( 'NONE', ( #79139, #116545, #27547, #82547 ) ) ;
#4200=VECTOR ( 'NONE', #72995, 1000.000000000000000 ) ;
#4201=ADVANCED_FACE ( 'NONE', ( #70809 ), #72705, .T. ) ;
#4202=DIRECTION ( 'NONE',  ( 0.000000000000000000, 1.000000000000000000, 0.000000000000000000 ) ) ;
#4203=ADVANCED_FACE ( 'NONE', ( #51190 ), #91575, .T. ) ;
#4204=AXIS2_PLACEMENT_3D ( 'NONE', #1181, #122259, #91494 ) ;
#4205=ORIENTED_EDGE ( 'NONE', *, *, #29732, .F. ) ;
#4206=ORIENTED_EDGE ( 'NONE', *, *, #1401, .T. ) ;
#4207=EDGE_CURVE ( 'NONE', #95831, #57530, #10010, .T. ) ;
#4208=ADVANCED_FACE ( 'NONE', ( #50520 ), #66432, .T. ) ;
#4209=VECTOR ( 'NONE', #13300, 1000.000000000000000 ) ;
#4211=CARTESIAN_POINT ( 'NONE',  ( 12.07106445316801846, -2.499999999999745981, 8.629160867383669498 ) ) ;
#4212=LINE ( 'NONE', #123997, #16533 ) ;
#4213=DIRECTION ( 'NONE',  ( -4.274815082592931898E-19, -0.9999939076577903929, -0.003490651415223739937 ) ) ;
#4214=EDGE_CURVE ( 'NONE', #16687, #89315, #60989, .T. ) ;
#4215=ADVANCED_FACE ( 'NONE', ( #112032 ), #60201, .T. ) ;
#4216=EDGE_LOOP ( 'NONE', ( #23715, #93666 ) ) ;
#4217=DIRECTION ( 'NONE',  ( -0.000000000000000000, 1.000000000000000000, -0.000000000000000000 ) ) ;
#4218=EDGE_CURVE ( 'NONE', #64387, #112983, #87352, .T. ) ;
#4219=CONICAL_SURFACE ( 'NONE', #16726, 0.1000000000000000056, 0.003490658503988666988 ) ;
#4220=ADVANCED_FACE ( 'NONE', ( #99638 ), #39453, .T. ) ;
#4221=EDGE_LOOP ( 'NONE', ( #55316, #97115 ) ) ;
#4222=EDGE_CURVE ( 'NONE', #41353, #123277, #11233, .T. ) ;
#4223=ORIENTED_EDGE ( 'NONE', *, *, #40290, .F. ) ;
#4224=CARTESIAN_POINT ( 'NONE',  ( -2.050000000000033129, 12.50000000000000000, 6.495190528383297135 ) ) ;
#4225=EDGE_LOOP ( 'NONE', ( #113010, #83024, #74227, #78648 ) ) ;
#4226=DIRECTION ( 'NONE',  ( 0.000000000000000000, 0.000000000000000000, 1.000000000000000000 ) ) ;
#4227=ORIENTED_EDGE ( 'NONE', *, *, #73166, .F. ) ;
#4228=EDGE_CURVE ( 'NONE', #123416, #62801, #114543, .T. ) ;
#4229=DIRECTION ( 'NONE',  ( 0.000000000000000000, -0.000000000000000000, 1.000000000000000000 ) ) ;
#4230=CARTESIAN_POINT ( 'NONE',  ( 11.84999999999990727, 2.500000000000000000, -2.511473670974877948 ) ) ;
#4231=CARTESIAN_POINT ( 'NONE',  ( -11.04999999999999893, 2.500000000000000000, 6.248780366869520542 ) ) ;
#4232=DIRECTION ( 'NONE',  ( -4.274815082592931898E-19, -0.9999939076577903929, -0.003490651415223739937 ) ) ;
#4233=DIRECTION ( 'NONE',  ( -0.000000000000000000, 1.000000000000000000, -0.000000000000000000 ) ) ;
#4234=ORIENTED_EDGE ( 'NONE', *, *, #126215, .T. ) ;
#4235=DIRECTION ( 'NONE',  ( 0.000000000000000000, 0.000000000000000000, 1.000000000000000000 ) ) ;
#4236=VECTOR ( 'NONE', #5837, 1000.000000000000000 ) ;
#4237=AXIS2_PLACEMENT_3D ( 'NONE', #71882, #98734, #30025 ) ;
#4238=ORIENTED_EDGE ( 'NONE', *, *, #68714, .T. ) ;
#4239=CARTESIAN_POINT ( 'NONE',  ( -2.700000000000030376, 2.500000000000000000, 3.983716857408420964 ) ) ;
#4240=VERTEX_POINT ( 'NONE', #31537 ) ;
#4241=CARTESIAN_POINT ( 'NONE',  ( -4.600000000000028066, 2.500000000000000000, -3.537306695894649966 ) ) ;
#4242=LINE ( 'NONE', #44181, #55314 ) ;
#4243=FACE_OUTER_BOUND ( 'NONE', #97825, .T. ) ;
#4244=DIRECTION ( 'NONE',  ( 0.000000000000000000, 1.000000000000000000, 0.000000000000000000 ) ) ;
#4245=ORIENTED_EDGE ( 'NONE', *, *, #8216, .F. ) ;
#4246=DIRECTION ( 'NONE',  ( 0.000000000000000000, -0.000000000000000000, 1.000000000000000000 ) ) ;
#4247=VERTEX_POINT ( 'NONE', #71443 ) ;
#4248=ORIENTED_EDGE ( 'NONE', *, *, #106557, .T. ) ;
#4249=VERTEX_POINT ( 'NONE', #111359 ) ;
#4250=CARTESIAN_POINT ( 'NONE',  ( -6.050000000000022027, 2.500000000000000000, -1.818653347947326138 ) ) ;
#4251=DIRECTION ( 'NONE',  ( 0.000000000000000000, 1.000000000000000000, 0.000000000000000000 ) ) ;
#4253=DIRECTION ( 'NONE',  ( 0.000000000000000000, 0.000000000000000000, 1.000000000000000000 ) ) ;
#4254=CONICAL_SURFACE ( 'NONE', #60722, 0.09999999999999999167, 0.003490658503988666988 ) ;
#4255=CIRCLE ( 'NONE', #31476, 0.06509327318403745899 ) ;
#4256=CARTESIAN_POINT ( 'NONE',  ( -1.850000000000033396, 2.500000000000000000, -6.148780366869526226 ) ) ;
#4257=EDGE_CURVE ( 'NONE', #84067, #50060, #76906, .T. ) ;
#4258=CARTESIAN_POINT ( 'NONE',  ( -3.150000000000030109, 2.500000000000000000, -2.511473670974877948 ) ) ;
#4259=AXIS2_PLACEMENT_3D ( 'NONE', #32039, #111201, #73872 ) ;
#4260=VERTEX_POINT ( 'NONE', #109449 ) ;
#4261=DIRECTION ( 'NONE',  ( -0.000000000000000000, 1.000000000000000000, -0.000000000000000000 ) ) ;
#4262=VERTEX_POINT ( 'NONE', #59732 ) ;
#4263=CONICAL_SURFACE ( 'NONE', #58679, 0.1000000000000002554, 0.003490658503988666988 ) ;
#4264=DIRECTION ( 'NONE',  ( 0.000000000000000000, 1.000000000000000000, 0.000000000000000000 ) ) ;
#4265=EDGE_CURVE ( 'NONE', #41760, #70628, #62250, .T. ) ;
#4266=CARTESIAN_POINT ( 'NONE',  ( 1.049999999999954525, 2.500000000000000000, 1.918653347947321564 ) ) ;
#4267=PLANE ( 'NONE',  #15048 ) ;
#4268=CARTESIAN_POINT ( 'NONE',  ( -7.700000000000010836, 12.50000000000000000, 4.048810130592458201 ) ) ;
#4269=ORIENTED_EDGE ( 'NONE', *, *, #43968, .F. ) ;
#4270=CARTESIAN_POINT ( 'NONE',  ( -3.950000000000028155, 2.500000000000000000, -6.741600689897077281 ) ) ;
#4271=CARTESIAN_POINT ( 'NONE',  ( -10.40000000000000213, 2.500000000000000000, -2.276824562219559311E-15 ) ) ;
#4272=ORIENTED_EDGE ( 'NONE', *, *, #82245, .F. ) ;
#4273=EDGE_LOOP ( 'NONE', ( #110406, #64430 ) ) ;
#4274=DIRECTION ( 'NONE',  ( -0.000000000000000000, -1.000000000000000000, -0.000000000000000000 ) ) ;
#4275=VERTEX_POINT ( 'NONE', #117001 ) ;
#4276=EDGE_LOOP ( 'NONE', ( #96480, #68958 ) ) ;
#4277=CARTESIAN_POINT ( 'NONE',  ( -2.300000000000033573, 2.500000000000000000, 4.676537180435972552 ) ) ;
#4278=CIRCLE ( 'NONE', #113058, 0.1000000000000002554 ) ;
#4279=CIRCLE ( 'NONE', #18965, 0.06509327318403745899 ) ;
#4280=ORIENTED_EDGE ( 'NONE', *, *, #128761, .T. ) ;
#4281=CARTESIAN_POINT ( 'NONE',  ( -7.950000000000016165, 12.50000000000000000, -6.495190528383297135 ) ) ;
#4282=DIRECTION ( 'NONE',  ( 0.000000000000000000, 1.000000000000000000, 0.000000000000000000 ) ) ;
#4283=CARTESIAN_POINT ( 'NONE',  ( 5.399999999999933742, 2.500000000000000000, -0.1000000000000023925 ) ) ;
#4284=VERTEX_POINT ( 'NONE', #65987 ) ;
#4285=EDGE_CURVE ( 'NONE', #54835, #43630, #45620, .T. ) ;
#4286=AXIS2_PLACEMENT_3D ( 'NONE', #68856, #60351, #108773 ) ;
#4287=CARTESIAN_POINT ( 'NONE',  ( -8.550000000000013145, 2.500000000000000000, -1.918653347947326004 ) ) ;
#4288=LINE ( 'NONE', #104450, #3483 ) ;
#4289=VERTEX_POINT ( 'NONE', #115725 ) ;
#4290=DIRECTION ( 'NONE',  ( 0.000000000000000000, -0.9999939076577903929, 0.003490651415223739937 ) ) ;
#4291=FACE_OUTER_BOUND ( 'NONE', #120303, .T. ) ;
#4292=EDGE_CURVE ( 'NONE', #115818, #119776, #26075, .T. ) ;
#4293=EDGE_LOOP ( 'NONE', ( #6740, #126868, #41678, #103241 ) ) ;
#4294=ORIENTED_EDGE ( 'NONE', *, *, #57130, .T. ) ;
#4295=ORIENTED_EDGE ( 'NONE', *, *, #4356, .T. ) ;
#4296=PLANE ( 'NONE',  #108997 ) ;
#4297=CARTESIAN_POINT ( 'NONE',  ( 4.913542845176413820, 1.499999999999745981, 9.942462991075640133 ) ) ;
#4298=EDGE_CURVE ( 'NONE', #55110, #22492, #5776, .T. ) ;
#4299=ADVANCED_FACE ( 'NONE', ( #96724 ), #58137, .T. ) ;
#4300=CARTESIAN_POINT ( 'NONE',  ( -13.54999999999999005, 2.500000000000000000, -1.718653347947323828 ) ) ;
#4301=EDGE_CURVE ( 'NONE', #122300, #10500, #33486, .T. ) ;
#4302=FACE_BOUND ( 'NONE', #108885, .T. ) ;
#4303=ORIENTED_EDGE ( 'NONE', *, *, #4156, .T. ) ;
#4304=ADVANCED_FACE ( 'NONE', ( #16220 ), #106551, .T. ) ;
#4306=EDGE_CURVE ( 'NONE', #116514, #30053, #112420, .T. ) ;
#4307=DIRECTION ( 'NONE',  ( 0.000000000000000000, 0.000000000000000000, 1.000000000000000000 ) ) ;
#4308=CARTESIAN_POINT ( 'NONE',  ( 6.249999999999930722, 2.500000000000000000, 1.472243186433545459 ) ) ;
#4309=CARTESIAN_POINT ( 'NONE',  ( -6.450000000000017941, 2.500000000000000000, -6.741600689897077281 ) ) ;
#4310=DIRECTION ( 'NONE',  ( 0.000000000000000000, 1.000000000000000000, 0.000000000000000000 ) ) ;
#4311=EDGE_CURVE ( 'NONE', #128555, #22839, #53116, .T. ) ;
#4312=DIRECTION ( 'NONE',  ( -4.274815082592931898E-19, -0.9999939076577903929, -0.003490651415223739937 ) ) ;
#4313=EDGE_CURVE ( 'NONE', #30210, #33390, #129168, .T. ) ;
#4314=AXIS2_PLACEMENT_3D ( 'NONE', #31490, #32795, #110050 ) ;
#4315=ADVANCED_FACE ( 'NONE', ( #3363 ), #122883, .T. ) ;
#4316=VECTOR ( 'NONE', #129530, 1000.000000000000000 ) ;
#4317=FACE_OUTER_BOUND ( 'NONE', #42845, .T. ) ;
#4318=ORIENTED_EDGE ( 'NONE', *, *, #127317, .F. ) ;
#4319=EDGE_LOOP ( 'NONE', ( #124447, #94891, #76695, #79785 ) ) ;
#4320=ORIENTED_EDGE ( 'NONE', *, *, #74363, .T. ) ;
#4321=ORIENTED_EDGE ( 'NONE', *, *, #36425, .T. ) ;
#4322=ORIENTED_EDGE ( 'NONE', *, *, #108668, .T. ) ;
#4323=DIRECTION ( 'NONE',  ( 0.000000000000000000, 1.000000000000000000, 0.000000000000000000 ) ) ;
#4324=DIRECTION ( 'NONE',  ( 0.000000000000000000, 0.000000000000000000, 1.000000000000000000 ) ) ;
#4325=EDGE_LOOP ( 'NONE', ( #10689, #112272, #51009, #44829 ) ) ;
#4326=FACE_BOUND ( 'NONE', #14880, .T. ) ;
#4327=AXIS2_PLACEMENT_3D ( 'NONE', #44232, #52769, #64520 ) ;
#4328=DIRECTION ( 'NONE',  ( 0.000000000000000000, 0.000000000000000000, 1.000000000000000000 ) ) ;
#4329=DIRECTION ( 'NONE',  ( -0.000000000000000000, 1.000000000000000000, -0.000000000000000000 ) ) ;
#4331=CARTESIAN_POINT ( 'NONE',  ( 4.799999999999935874, 12.50000000000000000, 0.4115034346978109769 ) ) ;
#4332=FACE_OUTER_BOUND ( 'NONE', #78132, .T. ) ;
#4333=CARTESIAN_POINT ( 'NONE',  ( -6.850000000000017408, 12.50000000000000000, -2.511473670974877948 ) ) ;
#4334=ORIENTED_EDGE ( 'NONE', *, *, #60248, .T. ) ;
#4335=CARTESIAN_POINT ( 'NONE',  ( -1.900000000000034994, 2.500000000000000000, -0.3464101615137783474 ) ) ;
#4336=CIRCLE ( 'NONE', #94249, 0.06509327318403741736 ) ;
#4337=VERTEX_POINT ( 'NONE', #72751 ) ;
#4338=AXIS2_PLACEMENT_3D ( 'NONE', #107187, #77098, #129449 ) ;
#4339=ORIENTED_EDGE ( 'NONE', *, *, #88997, .T. ) ;
#4340=VERTEX_POINT ( 'NONE', #105272 ) ;
#4341=CARTESIAN_POINT ( 'NONE',  ( 12.89999999999990266, 12.50000000000000000, -5.022947341949754119 ) ) ;
#4342=CARTESIAN_POINT ( 'NONE',  ( 1.249999999999950262, 2.500000000000000000, 7.288010851410849256 ) ) ;
#4343=DIRECTION ( 'NONE',  ( -4.274815082592931898E-19, -0.9999939076577903929, -0.003490651415223739937 ) ) ;
#4344=ORIENTED_EDGE ( 'NONE', *, *, #27666, .T. ) ;
#4345=FACE_OUTER_BOUND ( 'NONE', #102561, .T. ) ;
#4346=CIRCLE ( 'NONE', #123497, 0.1000000000000002554 ) ;
#4347=DIRECTION ( 'NONE',  ( 0.000000000000000000, 1.000000000000000000, 0.000000000000000000 ) ) ;
#4348=CARTESIAN_POINT ( 'NONE',  ( 8.749999999999918288, 2.500000000000000000, -1.372243186433550033 ) ) ;
#4349=CIRCLE ( 'NONE', #75475, 0.1000000000000002554 ) ;
#4351=VERTEX_POINT ( 'NONE', #36552 ) ;
#4352=DIRECTION ( 'NONE',  ( 0.000000000000000000, -0.9999939076577903929, 0.003490651415223739937 ) ) ;
#4353=EDGE_CURVE ( 'NONE', #96180, #83282, #14190, .T. ) ;
#4354=ORIENTED_EDGE ( 'NONE', *, *, #267, .F. ) ;
#4355=DIRECTION ( 'NONE',  ( 0.000000000000000000, -0.9999939076577903929, 0.003490651415223739937 ) ) ;
#4356=EDGE_CURVE ( 'NONE', #94541, #32372, #37210, .T. ) ;
#4357=EDGE_LOOP ( 'NONE', ( #61401, #44400, #67231, #106963 ) ) ;
#4358=EDGE_CURVE ( 'NONE', #76656, #82327, #70642, .T. ) ;
#4359=EDGE_LOOP ( 'NONE', ( #62859, #24151, #94788, #123351 ) ) ;
#4360=CARTESIAN_POINT ( 'NONE',  ( 6.249999999999932498, 2.500000000000000000, -5.802370205355749988 ) ) ;
#4361=CARTESIAN_POINT ( 'NONE',  ( -1.250000000000035749, 12.50000000000000000, -7.188010851410854052 ) ) ;
#4362=FACE_OUTER_BOUND ( 'NONE', #11896, .T. ) ;
#4363=DIRECTION ( 'NONE',  ( 0.000000000000000000, 0.000000000000000000, 1.000000000000000000 ) ) ;
#4365=ORIENTED_EDGE ( 'NONE', *, *, #44552, .F. ) ;
#4366=EDGE_CURVE ( 'NONE', #122261, #70779, #49735, .T. ) ;
#4367=VERTEX_POINT ( 'NONE', #95456 ) ;
#4368=DIRECTION ( 'NONE',  ( -0.000000000000000000, -1.000000000000000000, -0.000000000000000000 ) ) ;
#4369=B_SPLINE_CURVE_WITH_KNOTS ( 'NONE', 3,
 ( #24216, #111960, #44489, #71361 ),
 .UNSPECIFIED., .F., .F.,
 ( 4, 4 ),
 ( 0.001845843513054588620, 0.003313552284081257640 ),
 .UNSPECIFIED. ) ;
#4370=DIRECTION ( 'NONE',  ( 0.000000000000000000, 0.000000000000000000, 1.000000000000000000 ) ) ;
#4371=CIRCLE ( 'NONE', #108852, 0.1000000000000002554 ) ;
#4372=CARTESIAN_POINT ( 'NONE',  ( -7.300000000000014921, 2.500000000000000000, 4.776537180435972196 ) ) ;
#4373=EDGE_LOOP ( 'NONE', ( #80647, #126471 ) ) ;
#4374=EDGE_LOOP ( 'NONE', ( #94410, #100301, #71815, #118820 ) ) ;
#4375=AXIS2_PLACEMENT_3D ( 'NONE', #64314, #73480, #83942 ) ;
#4376=CARTESIAN_POINT ( 'NONE',  ( -8.550000000000013145, 12.50000000000000000, -1.818653347947326138 ) ) ;
#4377=EDGE_LOOP ( 'NONE', ( #124922, #73462, #112230, #106261 ) ) ;
#4378=PLANE ( 'NONE',  #62505 ) ;
#4379=CIRCLE ( 'NONE', #83820, 0.06509327318403745899 ) ;
#4380=DIRECTION ( 'NONE',  ( 0.000000000000000000, -0.9999939076577903929, 0.003490651415223739937 ) ) ;
#4381=VERTEX_POINT ( 'NONE', #85626 ) ;
#4382=DIRECTION ( 'NONE',  ( -0.000000000000000000, -1.000000000000000000, -0.000000000000000000 ) ) ;
#4383=DIRECTION ( 'NONE',  ( 0.000000000000000000, 0.000000000000000000, -1.000000000000000000 ) ) ;
#4384=DIRECTION ( 'NONE',  ( 0.000000000000000000, 1.000000000000000000, 0.000000000000000000 ) ) ;
#4385=AXIS2_PLACEMENT_3D ( 'NONE', #8252, #48188, #108392 ) ;
#4386=ADVANCED_FACE ( 'NONE', ( #77106 ), #99900, .T. ) ;
#4387=CARTESIAN_POINT ( 'NONE',  ( 1.449999999999951328, 12.50000000000000000, -1.818653347947326138 ) ) ;
#4388=ORIENTED_EDGE ( 'NONE', *, *, #32501, .T. ) ;
#4389=DIRECTION ( 'NONE',  ( 0.000000000000000000, -0.9999939076577903929, 0.003490651415223739937 ) ) ;
#4390=CARTESIAN_POINT ( 'NONE',  ( 65.40763333624980191, -3.109051995112019906, 5.794606894455887058 ) ) ;
#4391=VERTEX_POINT ( 'NONE', #102216 ) ;
#4392=ORIENTED_EDGE ( 'NONE', *, *, #30655, .T. ) ;
#4394=DIRECTION ( 'NONE',  ( 0.000000000000000000, 0.000000000000000000, 1.000000000000000000 ) ) ;
#4395=DIRECTION ( 'NONE',  ( 0.000000000000000000, 1.000000000000000000, 0.000000000000000000 ) ) ;
#4396=CARTESIAN_POINT ( 'NONE',  ( 12.09999999999990550, 12.50000000000000000, -4.330127018922201643 ) ) ;
#4397=CARTESIAN_POINT ( 'NONE',  ( -13.94999999999998685, 12.50000000000000000, 1.818653347947325472 ) ) ;
#4398=CIRCLE ( 'NONE', #88025, 0.09999999999999982514 ) ;
#4399=CARTESIAN_POINT ( 'NONE',  ( -10.40000000000000213, 12.50000000000000000, 3.702399969078682407 ) ) ;
#4400=CARTESIAN_POINT ( 'NONE',  ( 12.29999999999990479, 2.500000000000000000, 4.576537180435972019 ) ) ;
#4401=EDGE_CURVE ( 'NONE', #87296, #124884, #53919, .T. ) ;
#4402=CARTESIAN_POINT ( 'NONE',  ( 10.59999999999990905, 2.500000000000000000, -3.983716857408426293 ) ) ;
#4403=DIRECTION ( 'NONE',  ( 0.000000000000000000, 0.000000000000000000, 1.000000000000000000 ) ) ;
#4405=DIRECTION ( 'NONE',  ( -4.274815082592931898E-19, -0.9999939076577903929, -0.003490651415223739937 ) ) ;
#4406=VECTOR ( 'NONE', #106028, 1000.000000000000000 ) ;
#4407=ORIENTED_EDGE ( 'NONE', *, *, #79092, .T. ) ;
#4408=CIRCLE ( 'NONE', #31544, 0.06509327318403745899 ) ;
#4409=VERTEX_POINT ( 'NONE', #32842 ) ;
#4410=ORIENTED_EDGE ( 'NONE', *, *, #94442, .F. ) ;
#4411=ORIENTED_EDGE ( 'NONE', *, *, #18673, .T. ) ;
#4412=EDGE_CURVE ( 'NONE', #107061, #31226, #23009, .T. ) ;
#4413=DIRECTION ( 'NONE',  ( 0.000000000000000000, 0.000000000000000000, 1.000000000000000000 ) ) ;
#4414=DIRECTION ( 'NONE',  ( 0.000000000000000000, 0.000000000000000000, 1.000000000000000000 ) ) ;
#4415=LINE ( 'NONE', #5082, #75018 ) ;
#4416=AXIS2_PLACEMENT_3D ( 'NONE', #70271, #70916, #51295 ) ;
#4417=CIRCLE ( 'NONE', #115138, 0.06509327318403745899 ) ;
#4418=ORIENTED_EDGE ( 'NONE', *, *, #4158, .F. ) ;
#4419=CARTESIAN_POINT ( 'NONE',  ( -17.50000000000000000, -1.500000000000000000, -8.999999999999998224 ) ) ;
#4420=FACE_OUTER_BOUND ( 'NONE', #61689, .T. ) ;
#4421=CARTESIAN_POINT ( 'NONE',  ( -8.950000000000008171, 12.50000000000000000, 1.818653347947321475 ) ) ;
#4422=ORIENTED_EDGE ( 'NONE', *, *, #22963, .T. ) ;
#4423=CARTESIAN_POINT ( 'NONE',  ( 10.19999999999991225, 2.500000000000000000, 4.083716857408420609 ) ) ;
#4424=LINE ( 'NONE', #26679, #35381 ) ;
#4425=EDGE_LOOP ( 'NONE', ( #5466, #113025, #26453, #60792 ) ) ;
#4426=VECTOR ( 'NONE', #42170, 1000.000000000000000 ) ;
#4427=ORIENTED_EDGE ( 'NONE', *, *, #108363, .T. ) ;
#4428=EDGE_LOOP ( 'NONE', ( #103505, #74131, #27819, #29604 ) ) ;
#4429=ORIENTED_EDGE ( 'NONE', *, *, #23159, .F. ) ;
#4430=CARTESIAN_POINT ( 'NONE',  ( -1.250000000000035749, 2.500000000000000000, -7.188010851410854052 ) ) ;
#4431=AXIS2_PLACEMENT_3D ( 'NONE', #21389, #120880, #22058 ) ;
#4432=DIRECTION ( 'NONE',  ( 0.000000000000000000, -0.9999939076577903929, 0.003490651415223739937 ) ) ;
#4433=CARTESIAN_POINT ( 'NONE',  ( 5.649999999999936406, 12.50000000000000000, -6.148780366869526226 ) ) ;
#4434=LINE ( 'NONE', #77079, #45737 ) ;
#4436=EDGE_CURVE ( 'NONE', #30658, #112113, #41423, .T. ) ;
#4437=CIRCLE ( 'NONE', #104796, 0.1000000000000002554 ) ;
#4438=AXIS2_PLACEMENT_3D ( 'NONE', #114995, #43085, #123532 ) ;
#4439=DIRECTION ( 'NONE',  ( 0.000000000000000000, 0.000000000000000000, 1.000000000000000000 ) ) ;
#4440=VERTEX_POINT ( 'NONE', #58754 ) ;
#4441=DIRECTION ( 'NONE',  ( 0.000000000000000000, 0.000000000000000000, -1.000000000000000000 ) ) ;
#4442=CARTESIAN_POINT ( 'NONE',  ( 11.74779829703483180, -2.500000000000000888, -7.682567037524495213 ) ) ;
#4443=DIRECTION ( 'NONE',  ( 0.000000000000000000, -0.9999939076577903929, 0.003490651415223739937 ) ) ;
#4444=CARTESIAN_POINT ( 'NONE',  ( 16.68526679984168481, -0.4774970013447560335, 5.954360761636621646 ) ) ;
#4445=ADVANCED_FACE ( 'NONE', ( #128140 ), #51876, .T. ) ;
#4446=ORIENTED_EDGE ( 'NONE', *, *, #105266, .T. ) ;
#4447=EDGE_LOOP ( 'NONE', ( #6404, #96028, #101084, #37992 ) ) ;
#4448=EDGE_LOOP ( 'NONE', ( #128476, #119347, #123915, #116100 ) ) ;
#4449=CARTESIAN_POINT ( 'NONE',  ( 1.699999999999950218, 2.500000000000000000, 4.430127018922196847 ) ) ;
#4450=LINE ( 'NONE', #65981, #33088 ) ;
#4451=ADVANCED_FACE ( 'NONE', ( #48942 ), #58118, .T. ) ;
#4452=EDGE_CURVE ( 'NONE', #17249, #127376, #79052, .T. ) ;
#4453=CARTESIAN_POINT ( 'NONE',  ( 9.149999999999920419, 12.50000000000000000, -5.802370205355749988 ) ) ;
#4454=ADVANCED_FACE ( 'NONE', ( #448 ), #34385, .T. ) ;
#4455=FACE_BOUND ( 'NONE', #48394, .T. ) ;
#4456=EDGE_CURVE ( 'NONE', #76524, #66544, #15474, .T. ) ;
#4457=CARTESIAN_POINT ( 'NONE',  ( 1.249999999999988454, 2.500000000000000000, -2.265063509461101798 ) ) ;
#4458=CARTESIAN_POINT ( 'NONE',  ( -0.4000000000000339950, 12.50000000000000000, 0.6928203230275518099 ) ) ;
#4459=DIRECTION ( 'NONE',  ( -4.274815082592931898E-19, -0.9999939076577903929, -0.003490651415223739937 ) ) ;
#4460=ADVANCED_FACE ( 'NONE', ( #120258 ), #48951, .T. ) ;
#4461=VECTOR ( 'NONE', #124850, 1000.000000000000000 ) ;
#4462=AXIS2_PLACEMENT_3D ( 'NONE', #60936, #100848, #30214 ) ;
#4464=AXIS2_PLACEMENT_3D ( 'NONE', #25170, #73622, #55922 ) ;
#4465=ADVANCED_FACE ( 'NONE', ( #39143 ), #99326, .T. ) ;
#4466=CARTESIAN_POINT ( 'NONE',  ( 11.44999999999991047, 2.500000000000000000, 6.148780366869520009 ) ) ;
#4468=DIRECTION ( 'NONE',  ( 0.000000000000000000, 0.000000000000000000, -1.000000000000000000 ) ) ;
#4469=ORIENTED_EDGE ( 'NONE', *, *, #8475, .F. ) ;
#4470=EDGE_CURVE ( 'NONE', #5985, #58914, #63611, .T. ) ;
#4471=AXIS2_PLACEMENT_3D ( 'NONE', #8479, #121031, #48420 ) ;
#4472=ADVANCED_FACE ( 'NONE', ( #48288 ), #38490, .T. ) ;
#4473=CARTESIAN_POINT ( 'NONE',  ( -2.500000000000030642, 12.50000000000000000, -5.088040615133791356 ) ) ;
#4474=CONICAL_SURFACE ( 'NONE', #127831, 0.09999999999999999167, 0.003490658503988666988 ) ;
#4475=ORIENTED_EDGE ( 'NONE', *, *, #80923, .T. ) ;
#4476=ORIENTED_EDGE ( 'NONE', *, *, #109244, .F. ) ;
#4477=ORIENTED_EDGE ( 'NONE', *, *, #17053, .T. ) ;
#4478=ORIENTED_EDGE ( 'NONE', *, *, #106902, .F. ) ;
#4479=DIRECTION ( 'NONE',  ( -0.000000000000000000, 1.000000000000000000, -0.000000000000000000 ) ) ;
#4480=FACE_BOUND ( 'NONE', #93709, .T. ) ;
#4481=EDGE_CURVE ( 'NONE', #127950, #35702, #20116, .T. ) ;
#4482=FACE_OUTER_BOUND ( 'NONE', #3109, .T. ) ;
#4483=EDGE_LOOP ( 'NONE', ( #23092, #86846, #75870, #45001 ) ) ;
#4484=CARTESIAN_POINT ( 'NONE',  ( 26.61818291006873949, 2.722754637269844569, 4.358315985293821804 ) ) ;
#4485=CARTESIAN_POINT ( 'NONE',  ( -0.4500000000000397571, 2.500000000000000000, -2.065063509461102065 ) ) ;
#4486=VERTEX_POINT ( 'NONE', #78410 ) ;
#4487=CARTESIAN_POINT ( 'NONE',  ( -9.600000000000008527, 12.50000000000000000, -2.385244779468109755E-15 ) ) ;
#4488=DIRECTION ( 'NONE',  ( -0.000000000000000000, 1.000000000000000000, -0.000000000000000000 ) ) ;
#4489=ORIENTED_EDGE ( 'NONE', *, *, #16331, .T. ) ;
#4490=DIRECTION ( 'NONE',  ( 0.000000000000000000, 0.000000000000000000, -1.000000000000000000 ) ) ;
#4491=CARTESIAN_POINT ( 'NONE',  ( -11.89999999999999680, 12.50000000000000000, -0.3464101615137741841 ) ) ;
#4492=CONICAL_SURFACE ( 'NONE', #8712, 0.1000000000000002554, 0.003490658503988666988 ) ;
#4493=VECTOR ( 'NONE', #89266, 1000.000000000000000 ) ;
#4494=VERTEX_POINT ( 'NONE', #10296 ) ;
#4495=CARTESIAN_POINT ( 'NONE',  ( 10.64999999999991331, 12.50000000000000000, -2.446380397790840266 ) ) ;
#4496=LINE ( 'NONE', #14332, #60292 ) ;
#4497=CARTESIAN_POINT ( 'NONE',  ( -11.44999999999999751, 2.500000000000000000, -6.841600689897074261 ) ) ;
#4498=ORIENTED_EDGE ( 'NONE', *, *, #2129, .T. ) ;
#4499=EDGE_LOOP ( 'NONE', ( #90852, #12131, #12803, #72787 ) ) ;
#4500=CARTESIAN_POINT ( 'NONE',  ( -8.749999999999976907, 2.500000000000000000, -6.595190528383296780 ) ) ;
#4501=AXIS2_PLACEMENT_3D ( 'NONE', #53592, #103333, #3206 ) ;
#4502=ORIENTED_EDGE ( 'NONE', *, *, #58072, .T. ) ;
#4503=LINE ( 'NONE', #16267, #49168 ) ;
#4504=AXIS2_PLACEMENT_3D ( 'NONE', #107939, #59519, #58220 ) ;
#4505=DIRECTION ( 'NONE',  ( -0.000000000000000000, -1.000000000000000000, -0.000000000000000000 ) ) ;
#4506=EDGE_CURVE ( 'NONE', #22468, #124086, #111639, .T. ) ;
#4507=ORIENTED_EDGE ( 'NONE', *, *, #127729, .T. ) ;
#4508=AXIS2_PLACEMENT_3D ( 'NONE', #88126, #36505, #126803 ) ;
#4509=CARTESIAN_POINT ( 'NONE',  ( 8.749999999999918288, 2.500000000000000000, 7.188010851410848723 ) ) ;
#4510=EDGE_CURVE ( 'NONE', #21203, #103425, #94910, .T. ) ;
#4511=DIRECTION ( 'NONE',  ( -0.000000000000000000, 1.000000000000000000, -0.000000000000000000 ) ) ;
#4512=CARTESIAN_POINT ( 'NONE',  ( -8.150000000000009237, 12.50000000000000000, 6.841600689897072485 ) ) ;
#4513=FACE_OUTER_BOUND ( 'NONE', #3866, .T. ) ;
#4516=CONICAL_SURFACE ( 'NONE', #65165, 0.1000000000000000056, 0.003490658503988666988 ) ;
#4517=ADVANCED_FACE ( 'NONE', ( #67918 ), #97056, .T. ) ;
#4518=ORIENTED_EDGE ( 'NONE', *, *, #16702, .F. ) ;
#4520=VERTEX_POINT ( 'NONE', #7700 ) ;
#4521=CARTESIAN_POINT ( 'NONE',  ( -3.350000000000029399, 2.500000000000000000, 6.395190528383296602 ) ) ;
#4522=DIRECTION ( 'NONE',  ( 0.000000000000000000, 0.000000000000000000, 1.000000000000000000 ) ) ;
#4523=VECTOR ( 'NONE', #413, 1000.000000000000000 ) ;
#4524=DIRECTION ( 'NONE',  ( -0.000000000000000000, 1.000000000000000000, -0.000000000000000000 ) ) ;
#4525=ORIENTED_EDGE ( 'NONE', *, *, #42184, .T. ) ;
#4526=ORIENTED_EDGE ( 'NONE', *, *, #24278, .F. ) ;
#4528=FACE_OUTER_BOUND ( 'NONE', #82693, .T. ) ;
#4529=AXIS2_PLACEMENT_3D ( 'NONE', #76298, #25910, #116205 ) ;
#4530=DIRECTION ( 'NONE',  ( 0.000000000000000000, 0.000000000000000000, 1.000000000000000000 ) ) ;
#4531=CARTESIAN_POINT ( 'NONE',  ( -8.950000000000009948, 2.500000000000000000, 2.411473670974873862 ) ) ;
#4532=DIRECTION ( 'NONE',  ( 0.000000000000000000, 1.000000000000000000, 0.000000000000000000 ) ) ;
#4533=AXIS2_PLACEMENT_3D ( 'NONE', #69779, #120814, #109716 ) ;
#4534=CARTESIAN_POINT ( 'NONE',  ( 8.549999999999920774, 2.500000000000000000, -2.611473670974877592 ) ) ;
#4535=DIRECTION ( 'NONE',  ( 0.000000000000000000, 1.000000000000000000, 0.000000000000000000 ) ) ;
#4536=CARTESIAN_POINT ( 'NONE',  ( -4.150000000000025224, 2.500000000000000000, 7.088010851410848190 ) ) ;
#4537=FACE_OUTER_BOUND ( 'NONE', #33821, .T. ) ;
#4538=DIRECTION ( 'NONE',  ( 0.000000000000000000, 0.000000000000000000, 1.000000000000000000 ) ) ;
#4539=ORIENTED_EDGE ( 'NONE', *, *, #116485, .T. ) ;
#4540=DIRECTION ( 'NONE',  ( 0.000000000000000000, 0.000000000000000000, 1.000000000000000000 ) ) ;
#4541=VERTEX_POINT ( 'NONE', #127499 ) ;
#4542=ORIENTED_EDGE ( 'NONE', *, *, #105893, .T. ) ;
#4543=CARTESIAN_POINT ( 'NONE',  ( -2.100000000000033396, 12.50000000000000000, 0.6277270498435120194 ) ) ;
#4544=CARTESIAN_POINT ( 'NONE',  ( -3.550000000000027356, 12.50000000000000000, 1.753560074763284016 ) ) ;
#4545=DIRECTION ( 'NONE',  ( -4.274815082592931898E-19, -0.9999939076577903929, -0.003490651415223739937 ) ) ;
#4546=EDGE_CURVE ( 'NONE', #88432, #17273, #124252, .T. ) ;
#4547=CARTESIAN_POINT ( 'NONE',  ( -4.550000000000022915, 2.500000000000000000, 2.265063509461097357 ) ) ;
#4548=FACE_OUTER_BOUND ( 'NONE', #104793, .T. ) ;
#4549=CARTESIAN_POINT ( 'NONE',  ( 2.899999999999945732, 12.50000000000000000, 0.06509327318403504425 ) ) ;
#4550=AXIS2_PLACEMENT_3D ( 'NONE', #91590, #12377, #52311 ) ;
#4551=CARTESIAN_POINT ( 'NONE',  ( 5.199999999999935341, 2.500000000000000000, -0.3464101615137783474 ) ) ;
#4552=ORIENTED_EDGE ( 'NONE', *, *, #20199, .F. ) ;
#4553=LINE ( 'NONE', #95555, #20406 ) ;
#4554=VECTOR ( 'NONE', #9597, 1000.000000000000000 ) ;
#4555=CIRCLE ( 'NONE', #100721, 0.1000000000000000472 ) ;
#4556=DIRECTION ( 'NONE',  ( 0.000000000000000000, 0.000000000000000000, 1.000000000000000000 ) ) ;
#4557=ORIENTED_EDGE ( 'NONE', *, *, #42678, .F. ) ;
#4559=ORIENTED_EDGE ( 'NONE', *, *, #94674, .F. ) ;
#4560=CIRCLE ( 'NONE', #21312, 0.09999999999999999167 ) ;
#4561=EDGE_LOOP ( 'NONE', ( #110918, #7485 ) ) ;
#4562=VECTOR ( 'NONE', #2272, 1000.000000000000000 ) ;
#4563=ADVANCED_FACE ( 'NONE', ( #30598 ), #82411, .T. ) ;
#4564=CIRCLE ( 'NONE', #12890, 0.06509327318403745899 ) ;
#4565=ADVANCED_FACE ( 'NONE', ( #60697 ), #101174, .T. ) ;
#4566=VERTEX_POINT ( 'NONE', #32534 ) ;
#4567=CARTESIAN_POINT ( 'NONE',  ( -10.65000000000000213, 2.500000000000000000, 2.511473670974873507 ) ) ;
#4568=CARTESIAN_POINT ( 'NONE',  ( -6.250000000000021316, 12.50000000000000000, -1.472243186433550122 ) ) ;
#4569=VECTOR ( 'NONE', #26578, 1000.000000000000000 ) ;
#4570=CARTESIAN_POINT ( 'NONE',  ( -14.14999999999998792, 2.500000000000000000, 2.957883832488652942 ) ) ;
#4571=CARTESIAN_POINT ( 'NONE',  ( 3.149999999999946176, 12.50000000000000000, -2.511473670974877948 ) ) ;
#4572=CARTESIAN_POINT ( 'NONE',  ( -14.34999999999998543, 12.50000000000000000, 2.446380397790839822 ) ) ;
#4573=ORIENTED_EDGE ( 'NONE', *, *, #29482, .F. ) ;
#4574=CARTESIAN_POINT ( 'NONE',  ( 76.44859290207541846, -3.583118647509688781, 6.086777568259361004 ) ) ;
#4575=ADVANCED_FACE ( 'NONE', ( #92062 ), #88648, .T. ) ;
#4576=PLANE ( 'NONE',  #9702 ) ;
#4577=DIRECTION ( 'NONE',  ( 0.000000000000000000, 0.000000000000000000, 1.000000000000000000 ) ) ;
#4578=ORIENTED_EDGE ( 'NONE', *, *, #62783, .T. ) ;
#4579=ORIENTED_EDGE ( 'NONE', *, *, #81077, .F. ) ;
#4580=ORIENTED_EDGE ( 'NONE', *, *, #62458, .T. ) ;
#4581=DIRECTION ( 'NONE',  ( -0.000000000000000000, 1.000000000000000000, -0.000000000000000000 ) ) ;
#4582=DIRECTION ( 'NONE',  ( -0.000000000000000000, -1.000000000000000000, -0.000000000000000000 ) ) ;
#4583=AXIS2_PLACEMENT_3D ( 'NONE', #128762, #100554, #61937 ) ;
#4585=VECTOR ( 'NONE', #115990, 1000.000000000000000 ) ;
#4586=ORIENTED_EDGE ( 'NONE', *, *, #25448, .F. ) ;
#4587=CARTESIAN_POINT ( 'NONE',  ( -7.950000000000009059, 2.500000000000000000, 6.495190528383297135 ) ) ;
#4588=CARTESIAN_POINT ( 'NONE',  ( -13.09999999999999254, 12.50000000000000000, -3.918623584224386391 ) ) ;
#4589=LINE ( 'NONE', #124409, #33746 ) ;
#4590=DIRECTION ( 'NONE',  ( 0.000000000000000000, -0.000000000000000000, 1.000000000000000000 ) ) ;
#4591=DIRECTION ( 'NONE',  ( 0.000000000000000000, -0.9999939076577903929, 0.003490651415223739937 ) ) ;
#4592=AXIS2_PLACEMENT_3D ( 'NONE', #111702, #82250, #72428 ) ;
#4593=AXIS2_PLACEMENT_3D ( 'NONE', #14046, #33090, #94548 ) ;
#4594=AXIS2_PLACEMENT_3D ( 'NONE', #95078, #84613, #36809 ) ;
#4595=EDGE_CURVE ( 'NONE', #11368, #63798, #32236, .T. ) ;
#4596=ORIENTED_EDGE ( 'NONE', *, *, #117838, .T. ) ;
#4597=DIRECTION ( 'NONE',  ( -0.000000000000000000, -1.000000000000000000, -0.000000000000000000 ) ) ;
#4598=CONICAL_SURFACE ( 'NONE', #29685, 0.09999999999999982514, 0.003490658503988666988 ) ;
#4599=ORIENTED_EDGE ( 'NONE', *, *, #57298, .F. ) ;
#4601=EDGE_CURVE ( 'NONE', #94495, #109058, #50866, .T. ) ;
#4603=DIRECTION ( 'NONE',  ( 0.000000000000000000, 0.000000000000000000, 1.000000000000000000 ) ) ;
#4604=EDGE_CURVE ( 'NONE', #117214, #126618, #59430, .T. ) ;
#4605=DIRECTION ( 'NONE',  ( 0.000000000000000000, 1.000000000000000000, 0.000000000000000000 ) ) ;
#4606=AXIS2_PLACEMENT_3D ( 'NONE', #11399, #90601, #50680 ) ;
#4607=DIRECTION ( 'NONE',  ( 0.000000000000000000, 0.000000000000000000, 1.000000000000000000 ) ) ;
#4608=CONICAL_SURFACE ( 'NONE', #117478, 0.09999999999999982514, 0.003490658503988666988 ) ;
#4609=DIRECTION ( 'NONE',  ( 0.000000000000000000, 0.000000000000000000, 1.000000000000000000 ) ) ;
#4610=EDGE_LOOP ( 'NONE', ( #18314, #54305, #72748, #62158 ) ) ;
#4611=CIRCLE ( 'NONE', #29696, 0.06509327318403745899 ) ;
#4612=CIRCLE ( 'NONE', #94527, 0.1000000000000002554 ) ;
#4613=CIRCLE ( 'NONE', #21370, 0.1000000000000000472 ) ;
#4614=ADVANCED_FACE ( 'NONE', ( #43638 ), #111042, .T. ) ;
#4615=EDGE_CURVE ( 'NONE', #108499, #29271, #55208, .T. ) ;
#4616=EDGE_LOOP ( 'NONE', ( #16262, #109759 ) ) ;
#4617=CARTESIAN_POINT ( 'NONE',  ( -4.999999999999990230, 12.50000000000000000, -4.330127018922201643 ) ) ;
#4618=CARTESIAN_POINT ( 'NONE',  ( -4.999999999999986677, 2.500000000000000000, -2.276824562219559311E-15 ) ) ;
#4619=EDGE_CURVE ( 'NONE', #42865, #59695, #81605, .T. ) ;
#4620=DIRECTION ( 'NONE',  ( -0.000000000000000000, 1.000000000000000000, -0.000000000000000000 ) ) ;
#4621=AXIS2_PLACEMENT_3D ( 'NONE', #10457, #20931, #8508 ) ;
#4622=FACE_OUTER_BOUND ( 'NONE', #57006, .T. ) ;
#4623=VERTEX_POINT ( 'NONE', #111716 ) ;
#4624=FACE_OUTER_BOUND ( 'NONE', #95766, .T. ) ;
#4625=EDGE_CURVE ( 'NONE', #128756, #75351, #13419, .T. ) ;
#4626=CARTESIAN_POINT ( 'NONE',  ( 2.699999999999947331, 2.500000000000000000, -4.776537180435978414 ) ) ;
#4627=AXIS2_PLACEMENT_3D ( 'NONE', #125573, #63453, #64089 ) ;
#4628=ORIENTED_EDGE ( 'NONE', *, *, #13066, .F. ) ;
#4629=DIRECTION ( 'NONE',  ( -0.000000000000000000, -1.000000000000000000, -0.000000000000000000 ) ) ;
#4630=EDGE_CURVE ( 'NONE', #25435, #109355, #92867, .T. ) ;
#4631=ORIENTED_EDGE ( 'NONE', *, *, #5367, .F. ) ;
#4632=EDGE_CURVE ( 'NONE', #61297, #68676, #103323, .T. ) ;
#4633=LINE ( 'NONE', #15091, #32856 ) ;
#4634=EDGE_LOOP ( 'NONE', ( #120322, #23997 ) ) ;
#4635=DIRECTION ( 'NONE',  ( -0.000000000000000000, -1.000000000000000000, -0.000000000000000000 ) ) ;
#4636=DIRECTION ( 'NONE',  ( -0.000000000000000000, -1.000000000000000000, -0.000000000000000000 ) ) ;
#4637=ORIENTED_EDGE ( 'NONE', *, *, #82218, .F. ) ;
#4638=EDGE_LOOP ( 'NONE', ( #73014, #91421 ) ) ;
#4641=DIRECTION ( 'NONE',  ( -0.000000000000000000, 1.000000000000000000, -0.000000000000000000 ) ) ;
#4642=VECTOR ( 'NONE', #84827, 1000.000000000000000 ) ;
#4643=DIRECTION ( 'NONE',  ( -4.274815082592931898E-19, -0.9999939076577903929, -0.003490651415223739937 ) ) ;
#4644=CARTESIAN_POINT ( 'NONE',  ( 9.999999999999914735, 2.500000000000000000, 0.6928203230275494784 ) ) ;
#4645=AXIS2_PLACEMENT_3D ( 'NONE', #90371, #25496, #2634 ) ;
#4646=DIRECTION ( 'NONE',  ( 0.000000000000000000, -0.000000000000000000, 1.000000000000000000 ) ) ;
#4647=DIRECTION ( 'NONE',  ( -0.000000000000000000, -1.000000000000000000, -0.000000000000000000 ) ) ;
#4648=AXIS2_PLACEMENT_3D ( 'NONE', #121639, #22184, #62101 ) ;
#4649=EDGE_LOOP ( 'NONE', ( #51158, #97507, #43525, #7560 ) ) ;
#4650=VECTOR ( 'NONE', #122417, 1000.000000000000000 ) ;
#4651=VERTEX_POINT ( 'NONE', #43007 ) ;
#4652=DIRECTION ( 'NONE',  ( -0.000000000000000000, 1.000000000000000000, -0.000000000000000000 ) ) ;
#4653=DIRECTION ( 'NONE',  ( -4.274815082592931898E-19, -0.9999939076577903929, -0.003490651415223739937 ) ) ;
#4654=DIRECTION ( 'NONE',  ( 0.000000000000000000, 0.000000000000000000, 1.000000000000000000 ) ) ;
#4655=CIRCLE ( 'NONE', #50660, 0.06509327318403745899 ) ;
#4656=DIRECTION ( 'NONE',  ( 0.000000000000000000, 1.000000000000000000, 0.000000000000000000 ) ) ;
#4657=VECTOR ( 'NONE', #67984, 1000.000000000000000 ) ;
#4658=ORIENTED_EDGE ( 'NONE', *, *, #50733, .F. ) ;
#4659=ORIENTED_EDGE ( 'NONE', *, *, #46653, .T. ) ;
#4660=DIRECTION ( 'NONE',  ( -0.000000000000000000, 1.000000000000000000, -0.000000000000000000 ) ) ;
#4661=ORIENTED_EDGE ( 'NONE', *, *, #117512, .F. ) ;
#4662=DIRECTION ( 'NONE',  ( 0.000000000000000000, 0.000000000000000000, -1.000000000000000000 ) ) ;
#4663=FACE_OUTER_BOUND ( 'NONE', #84560, .T. ) ;
#4664=AXIS2_PLACEMENT_3D ( 'NONE', #41164, #111821, #111142 ) ;
#4665=ORIENTED_EDGE ( 'NONE', *, *, #39109, .F. ) ;
#4666=FACE_OUTER_BOUND ( 'NONE', #91228, .T. ) ;
#4667=LINE ( 'NONE', #104809, #41091 ) ;
#4668=EDGE_CURVE ( 'NONE', #78495, #77492, #109587, .T. ) ;
#4669=DIRECTION ( 'NONE',  ( 0.000000000000000000, 0.000000000000000000, 1.000000000000000000 ) ) ;
#4670=CARTESIAN_POINT ( 'NONE',  ( -7.900000000000014566, 12.50000000000000000, -3.637306695894650055 ) ) ;
#4671=DIRECTION ( 'NONE',  ( -0.000000000000000000, -1.000000000000000000, -0.000000000000000000 ) ) ;
#4672=EDGE_CURVE ( 'NONE', #63967, #95786, #5009, .T. ) ;
#4673=DIRECTION ( 'NONE',  ( 0.000000000000000000, 0.000000000000000000, -1.000000000000000000 ) ) ;
#4675=CARTESIAN_POINT ( 'NONE',  ( 13.34999999999990017, 2.500000000000000000, 2.265063509461097357 ) ) ;
#4676=CARTESIAN_POINT ( 'NONE',  ( -8.750000000000010658, 12.50000000000000000, -7.188010851410848723 ) ) ;
#4677=CIRCLE ( 'NONE', #111292, 0.1000000000000002554 ) ;
#4678=ORIENTED_EDGE ( 'NONE', *, *, #24025, .T. ) ;
#4679=ORIENTED_EDGE ( 'NONE', *, *, #58409, .F. ) ;
#4680=VERTEX_POINT ( 'NONE', #63255 ) ;
#4681=CARTESIAN_POINT ( 'NONE',  ( -11.64999999999999680, 2.500000000000000000, -2.065063509461098068 ) ) ;
#4682=VERTEX_POINT ( 'NONE', #100592 ) ;
#4683=LINE ( 'NONE', #51421, #68647 ) ;
#4684=ORIENTED_EDGE ( 'NONE', *, *, #71147, .T. ) ;
#4685=EDGE_LOOP ( 'NONE', ( #106222, #124078, #127461, #68182 ) ) ;
#4686=ORIENTED_EDGE ( 'NONE', *, *, #122295, .F. ) ;
#4687=DIRECTION ( 'NONE',  ( 0.000000000000000000, 0.000000000000000000, 1.000000000000000000 ) ) ;
#4688=VECTOR ( 'NONE', #28459, 1000.000000000000000 ) ;
#4689=CONICAL_SURFACE ( 'NONE', #73748, 0.1000000000000002554, 0.003490658503988666988 ) ;
#4692=CARTESIAN_POINT ( 'NONE',  ( -0.6500000000000389910, 12.50000000000000000, -1.818653347947326138 ) ) ;
#4693=CARTESIAN_POINT ( 'NONE',  ( 7.299999999999926104, 2.500000000000000000, -3.983716857408426293 ) ) ;
#4694=CARTESIAN_POINT ( 'NONE',  ( 8.349999999999923261, 2.500000000000000000, -7.288010851410854585 ) ) ;
#4695=ORIENTED_EDGE ( 'NONE', *, *, #111015, .F. ) ;
#4696=AXIS2_PLACEMENT_3D ( 'NONE', #48123, #117458, #69685 ) ;
#4697=AXIS2_PLACEMENT_3D ( 'NONE', #17254, #18581, #76220 ) ;
#4698=DIRECTION ( 'NONE',  ( 0.000000000000000000, -0.9999939076577903929, 0.003490651415223739937 ) ) ;
#4699=ORIENTED_EDGE ( 'NONE', *, *, #9854, .F. ) ;
#4700=CONICAL_SURFACE ( 'NONE', #86176, 0.1000000000000000472, 0.003490658503988666988 ) ;
#4701=EDGE_LOOP ( 'NONE', ( #71112, #71264 ) ) ;
#4702=AXIS2_PLACEMENT_3D ( 'NONE', #52586, #2187, #82038 ) ;
#4703=ORIENTED_EDGE ( 'NONE', *, *, #8700, .F. ) ;
#4704=FACE_OUTER_BOUND ( 'NONE', #115315, .T. ) ;
#4705=EDGE_LOOP ( 'NONE', ( #103666, #45245, #41718, #89039 ) ) ;
#4706=ORIENTED_EDGE ( 'NONE', *, *, #120180, .F. ) ;
#4707=VERTEX_POINT ( 'NONE', #33176 ) ;
#4708=CIRCLE ( 'NONE', #56938, 0.1000000000000002554 ) ;
#4709=FACE_OUTER_BOUND ( 'NONE', #20776, .T. ) ;
#4710=CIRCLE ( 'NONE', #44448, 0.06509327318403745899 ) ;
#4711=EDGE_CURVE ( 'NONE', #84112, #70528, #20759, .T. ) ;
#4712=CARTESIAN_POINT ( 'NONE',  ( 11.89999999999990798, 2.500000000000000000, -3.983716857408426293 ) ) ;
#4713=FACE_OUTER_BOUND ( 'NONE', #129586, .T. ) ;
#4714=PLANE ( 'NONE',  #40101 ) ;
#4716=VECTOR ( 'NONE', #75249, 1000.000000000000000 ) ;
#4717=AXIS2_PLACEMENT_3D ( 'NONE', #74578, #104043, #5817 ) ;
#4718=DIRECTION ( 'NONE',  ( 0.000000000000000000, 1.000000000000000000, 0.000000000000000000 ) ) ;
#4719=ORIENTED_EDGE ( 'NONE', *, *, #127592, .F. ) ;
#4720=AXIS2_PLACEMENT_3D ( 'NONE', #84991, #16866, #126216 ) ;
#4721=DIRECTION ( 'NONE',  ( 0.000000000000000000, 1.000000000000000000, 0.000000000000000000 ) ) ;
#4722=ADVANCED_FACE ( 'NONE', ( #52154 ), #44839, .T. ) ;
#4723=ORIENTED_EDGE ( 'NONE', *, *, #110924, .T. ) ;
#4724=CARTESIAN_POINT ( 'NONE',  ( -8.550000000000013145, 2.500000000000000000, -6.741600689897072840 ) ) ;
#4725=EDGE_LOOP ( 'NONE', ( #81455, #30356, #1503, #107931 ) ) ;
#4726=CONICAL_SURFACE ( 'NONE', #94620, 0.1000000000000000472, 0.003490658503988666988 ) ;
#4727=DIRECTION ( 'NONE',  ( 0.000000000000000000, 0.000000000000000000, 1.000000000000000000 ) ) ;
#4728=VERTEX_POINT ( 'NONE', #41069 ) ;
#4729=ADVANCED_FACE ( 'NONE', ( #80972 ), #103833, .T. ) ;
#4730=ADVANCED_FACE ( 'NONE', ( #126028 ), #84822, .T. ) ;
#4731=ORIENTED_EDGE ( 'NONE', *, *, #64270, .F. ) ;
#4732=CARTESIAN_POINT ( 'NONE',  ( 4.349999999999941025, 12.50000000000000000, -1.753560074763288679 ) ) ;
#4733=FACE_OUTER_BOUND ( 'NONE', #31963, .T. ) ;
#4734=EDGE_CURVE ( 'NONE', #6533, #120460, #86093, .T. ) ;
#4735=FACE_OUTER_BOUND ( 'NONE', #104955, .T. ) ;
#4737=CARTESIAN_POINT ( 'NONE',  ( 10.84999999999991260, 12.50000000000000000, 5.802370205355744659 ) ) ;
#4738=ORIENTED_EDGE ( 'NONE', *, *, #120504, .T. ) ;
#4739=CARTESIAN_POINT ( 'NONE',  ( 3.749999999999944045, 12.50000000000000000, -2.857883832488653741 ) ) ;
#4740=CARTESIAN_POINT ( 'NONE',  ( 0.5999999999999547917, 2.500000000000000000, 4.083716857408420609 ) ) ;
#4741=VECTOR ( 'NONE', #45831, 1000.000000000000000 ) ;
#4742=EDGE_CURVE ( 'NONE', #63146, #33567, #120048, .T. ) ;
#4743=DIRECTION ( 'NONE',  ( 0.000000000000000000, -0.000000000000000000, 1.000000000000000000 ) ) ;
#4744=CARTESIAN_POINT ( 'NONE',  ( 17.50000000000000000, -2.500000000000000000, 2.922290670089274567 ) ) ;
#4745=CARTESIAN_POINT ( 'NONE',  ( -9.400000000000007461, 12.50000000000000000, 3.983716857408420076 ) ) ;
#4746=ORIENTED_EDGE ( 'NONE', *, *, #87661, .F. ) ;
#4747=CIRCLE ( 'NONE', #77918, 0.06509327318403745899 ) ;
#4748=EDGE_LOOP ( 'NONE', ( #55917, #32994 ) ) ;
#4749=CIRCLE ( 'NONE', #92503, 0.1000000000000002554 ) ;
#4750=CONICAL_SURFACE ( 'NONE', #23548, 0.1000000000000002554, 0.003490658503988666988 ) ;
#4751=ORIENTED_EDGE ( 'NONE', *, *, #39669, .T. ) ;
#4752=DIRECTION ( 'NONE',  ( -0.000000000000000000, -1.000000000000000000, -0.000000000000000000 ) ) ;
#4753=CARTESIAN_POINT ( 'NONE',  ( 11.24999999999991118, 12.50000000000000000, -2.792790559304616504 ) ) ;
#4754=AXIS2_PLACEMENT_3D ( 'NONE', #77823, #118400, #59518 ) ;
#4755=CIRCLE ( 'NONE', #77927, 0.1000000000000002554 ) ;
#4756=CIRCLE ( 'NONE', #71679, 0.1000000000000002554 ) ;
#4757=AXIS2_PLACEMENT_3D ( 'NONE', #5819, #123210, #86973 ) ;
#4758=CIRCLE ( 'NONE', #103078, 0.1000000000000000472 ) ;
#4760=LINE ( 'NONE', #125205, #28133 ) ;
#4761=LINE ( 'NONE', #104276, #113377 ) ;
#4762=DIRECTION ( 'NONE',  ( 0.000000000000000000, 0.000000000000000000, 1.000000000000000000 ) ) ;
#4763=CARTESIAN_POINT ( 'NONE',  ( 8.099999999999923261, 12.50000000000000000, 4.048810130592458201 ) ) ;
#4764=ORIENTED_EDGE ( 'NONE', *, *, #45432, .T. ) ;
#4765=DIRECTION ( 'NONE',  ( 0.000000000000000000, 1.000000000000000000, 0.000000000000000000 ) ) ;
#4766=EDGE_CURVE ( 'NONE', #16720, #68464, #28104, .T. ) ;
#4767=DIRECTION ( 'NONE',  ( 0.000000000000000000, 0.000000000000000000, -1.000000000000000000 ) ) ;
#4768=CARTESIAN_POINT ( 'NONE',  ( 14.34999999999989662, 2.500000000000000000, 2.511473670974873507 ) ) ;
#4769=ORIENTED_EDGE ( 'NONE', *, *, #64059, .T. ) ;
#4770=EDGE_CURVE ( 'NONE', #33245, #78150, #44746, .T. ) ;
#4771=EDGE_CURVE ( 'NONE', #86814, #39666, #78196, .T. ) ;
#4772=CARTESIAN_POINT ( 'NONE',  ( 15.59999999999988951, 2.500000000000000000, -0.3464101615137783474 ) ) ;
#4773=AXIS2_PLACEMENT_3D ( 'NONE', #110879, #61808, #49413 ) ;
#4774=EDGE_LOOP ( 'NONE', ( #65861, #105035, #118796, #52460 ) ) ;
#4775=FACE_OUTER_BOUND ( 'NONE', #110979, .T. ) ;
#4776=EDGE_CURVE ( 'NONE', #41506, #61373, #118070, .T. ) ;
#4777=EDGE_CURVE ( 'NONE', #55365, #93720, #14766, .T. ) ;
#4778=VERTEX_POINT ( 'NONE', #94005 ) ;
#4779=DIRECTION ( 'NONE',  ( 0.000000000000000000, 0.000000000000000000, 1.000000000000000000 ) ) ;
#4780=LINE ( 'NONE', #3519, #27875 ) ;
#4781=EDGE_CURVE ( 'NONE', #117938, #45123, #26049, .T. ) ;
#4782=DIRECTION ( 'NONE',  ( 0.000000000000000000, 0.000000000000000000, -1.000000000000000000 ) ) ;
#4783=ADVANCED_FACE ( 'NONE', ( #35107 ), #111722, .T. ) ;
#4784=CIRCLE ( 'NONE', #8996, 0.1000000000000002554 ) ;
#4785=ORIENTED_EDGE ( 'NONE', *, *, #97404, .F. ) ;
#4786=CIRCLE ( 'NONE', #59101, 0.09999999999999982514 ) ;
#4787=AXIS2_PLACEMENT_3D ( 'NONE', #70053, #117839, #107393 ) ;
#4789=EDGE_CURVE ( 'NONE', #117945, #125498, #24629, .T. ) ;
#4790=CARTESIAN_POINT ( 'NONE',  ( -11.89999999999999680, 12.50000000000000000, 0.3464101615137776813 ) ) ;
#4791=AXIS2_PLACEMENT_3D ( 'NONE', #98180, #18968, #70025 ) ;
#4792=VERTEX_POINT ( 'NONE', #85472 ) ;
#4793=AXIS2_PLACEMENT_3D ( 'NONE', #49680, #18896, #69948 ) ;
#4794=EDGE_CURVE ( 'NONE', #85654, #29791, #92958, .T. ) ;
#4795=DIRECTION ( 'NONE',  ( -0.000000000000000000, -1.000000000000000000, -0.000000000000000000 ) ) ;
#4796=AXIS2_PLACEMENT_3D ( 'NONE', #57675, #27539, #36101 ) ;
#4797=EDGE_CURVE ( 'NONE', #52060, #112457, #55294, .T. ) ;
#4798=VERTEX_POINT ( 'NONE', #114919 ) ;
#4799=ORIENTED_EDGE ( 'NONE', *, *, #120226, .T. ) ;
#4800=CARTESIAN_POINT ( 'NONE',  ( -8.150000000000012790, 2.500000000000000000, 2.511473670974873507 ) ) ;
#4801=DIRECTION ( 'NONE',  ( 0.000000000000000000, -0.000000000000000000, 1.000000000000000000 ) ) ;
#4802=VERTEX_POINT ( 'NONE', #25244 ) ;
#4803=DIRECTION ( 'NONE',  ( 0.000000000000000000, 0.000000000000000000, 1.000000000000000000 ) ) ;
#4804=DIRECTION ( 'NONE',  ( 0.000000000000000000, 0.000000000000000000, 1.000000000000000000 ) ) ;
#4805=CIRCLE ( 'NONE', #17316, 0.06509327318403745899 ) ;
#4806=VERTEX_POINT ( 'NONE', #115555 ) ;
#4807=CARTESIAN_POINT ( 'NONE',  ( -13.14999999999999147, 12.50000000000000000, -2.446380397790838046 ) ) ;
#4808=CARTESIAN_POINT ( 'NONE',  ( 6.649999999999930189, 12.50000000000000000, -1.407149913249512663 ) ) ;
#4809=AXIS2_PLACEMENT_3D ( 'NONE', #78905, #68409, #118804 ) ;
#4810=AXIS2_PLACEMENT_3D ( 'NONE', #81539, #102467, #109208 ) ;
#4811=CIRCLE ( 'NONE', #96852, 0.06509327318403745899 ) ;
#4812=DIRECTION ( 'NONE',  ( 0.000000000000000000, 1.000000000000000000, 0.000000000000000000 ) ) ;
#4813=FACE_OUTER_BOUND ( 'NONE', #26377, .T. ) ;
#4814=DIRECTION ( 'NONE',  ( 0.000000000000000000, 0.000000000000000000, 1.000000000000000000 ) ) ;
#4815=FACE_OUTER_BOUND ( 'NONE', #57206, .T. ) ;
#4816=AXIS2_PLACEMENT_3D ( 'NONE', #84844, #57326, #126051 ) ;
#4817=DIRECTION ( 'NONE',  ( 0.000000000000000000, 0.000000000000000000, 1.000000000000000000 ) ) ;
#4818=ORIENTED_EDGE ( 'NONE', *, *, #84146, .F. ) ;
#4819=CIRCLE ( 'NONE', #71749, 0.06509327318403745899 ) ;
#4820=ORIENTED_EDGE ( 'NONE', *, *, #326, .T. ) ;
#4821=ORIENTED_EDGE ( 'NONE', *, *, #40578, .T. ) ;
#4822=ORIENTED_EDGE ( 'NONE', *, *, #52211, .F. ) ;
#4824=DIRECTION ( 'NONE',  ( -0.000000000000000000, -1.000000000000000000, -0.000000000000000000 ) ) ;
#4825=DIRECTION ( 'NONE',  ( 0.000000000000000000, -0.000000000000000000, 1.000000000000000000 ) ) ;
#4826=VERTEX_POINT ( 'NONE', #65163 ) ;
#4827=FACE_BOUND ( 'NONE', #40551, .T. ) ;
#4828=DIRECTION ( 'NONE',  ( 0.000000000000000000, 0.000000000000000000, 1.000000000000000000 ) ) ;
#4829=DIRECTION ( 'NONE',  ( 0.000000000000000000, 0.000000000000000000, 1.000000000000000000 ) ) ;
#4830=DIRECTION ( 'NONE',  ( 0.000000000000000000, 1.000000000000000000, 0.000000000000000000 ) ) ;
#4831=ADVANCED_FACE ( 'NONE', ( #64540 ), #5102, .T. ) ;
#4832=FACE_OUTER_BOUND ( 'NONE', #58745, .T. ) ;
#4833=CARTESIAN_POINT ( 'NONE',  ( 3.349999999999945466, 2.500000000000000000, -6.495190528383302464 ) ) ;
#4834=CARTESIAN_POINT ( 'NONE',  ( 13.54999999999990123, 12.50000000000000000, 1.818653347947321475 ) ) ;
#4835=CARTESIAN_POINT ( 'NONE',  ( 3.549999999999940314, 2.500000000000000000, 6.941600689897073018 ) ) ;
#4836=DIRECTION ( 'NONE',  ( 0.000000000000000000, 1.000000000000000000, 0.000000000000000000 ) ) ;
#4837=AXIS2_PLACEMENT_3D ( 'NONE', #119672, #28735, #68643 ) ;
#4838=VECTOR ( 'NONE', #37079, 1000.000000000000000 ) ;
#4839=CARTESIAN_POINT ( 'NONE',  ( 5.799999999999933209, 12.50000000000000000, -0.06509327318403980434 ) ) ;
#4840=CARTESIAN_POINT ( 'NONE',  ( -13.14999999999999147, 2.500000000000000000, -1.818653347947323917 ) ) ;
#4841=EDGE_CURVE ( 'NONE', #62185, #4982, #56001, .T. ) ;
#4842=AXIS2_PLACEMENT_3D ( 'NONE', #77547, #98466, #127314 ) ;
#4843=EDGE_LOOP ( 'NONE', ( #38595, #62513, #109993, #82465 ) ) ;
#4844=ORIENTED_EDGE ( 'NONE', *, *, #73202, .T. ) ;
#4845=ORIENTED_EDGE ( 'NONE', *, *, #56074, .T. ) ;
#4846=AXIS2_PLACEMENT_3D ( 'NONE', #39943, #10463, #50390 ) ;
#4847=ORIENTED_EDGE ( 'NONE', *, *, #69909, .T. ) ;
#4848=CARTESIAN_POINT ( 'NONE',  ( 1.249999999999986899, 2.500000000000000000, 6.495190528383297135 ) ) ;
#4849=CIRCLE ( 'NONE', #19425, 0.1000000000000000472 ) ;
#4850=EDGE_LOOP ( 'NONE', ( #77696, #30667, #110011, #113770 ) ) ;
#4851=CIRCLE ( 'NONE', #90541, 0.06509327318403745899 ) ;
#4852=LINE ( 'NONE', #83445, #31886 ) ;
#4853=ORIENTED_EDGE ( 'NONE', *, *, #18506, .T. ) ;
#4854=ORIENTED_EDGE ( 'NONE', *, *, #85888, .T. ) ;
#4855=AXIS2_PLACEMENT_3D ( 'NONE', #109214, #66713, #7142 ) ;
#4856=AXIS2_PLACEMENT_3D ( 'NONE', #34580, #115035, #106515 ) ;
#4857=AXIS2_PLACEMENT_3D ( 'NONE', #48732, #29101, #89923 ) ;
#4858=CARTESIAN_POINT ( 'NONE',  ( 3.677269697637739476, -2.500000000000000444, 8.999999999915248239 ) ) ;
#4859=LINE ( 'NONE', #64433, #58347 ) ;
#4860=CARTESIAN_POINT ( 'NONE',  ( -3.350000000000029399, 2.500000000000000000, 6.495190528383297135 ) ) ;
#4861=DIRECTION ( 'NONE',  ( 0.000000000000000000, 0.000000000000000000, 1.000000000000000000 ) ) ;
#4862=AXIS2_PLACEMENT_3D ( 'NONE', #105529, #33575, #44036 ) ;
#4863=EDGE_LOOP ( 'NONE', ( #114614, #58454, #20937, #19980 ) ) ;
#4864=CIRCLE ( 'NONE', #88495, 0.06509327318403745899 ) ;
#4865=EDGE_LOOP ( 'NONE', ( #65689, #11282 ) ) ;
#4866=ORIENTED_EDGE ( 'NONE', *, *, #123504, .F. ) ;
#4867=CARTESIAN_POINT ( 'NONE',  ( 5.849999999999933031, 2.500000000000000000, -1.572243186433550211 ) ) ;
#4868=VERTEX_POINT ( 'NONE', #6244 ) ;
#4869=DIRECTION ( 'NONE',  ( 0.000000000000000000, 1.000000000000000000, 0.000000000000000000 ) ) ;
#4870=EDGE_LOOP ( 'NONE', ( #56891, #63140 ) ) ;
#4871=EDGE_LOOP ( 'NONE', ( #105938, #82775 ) ) ;
#4872=DIRECTION ( 'NONE',  ( 0.000000000000000000, 0.000000000000000000, -1.000000000000000000 ) ) ;
#4873=DIRECTION ( 'NONE',  ( 0.000000000000000000, 0.000000000000000000, 1.000000000000000000 ) ) ;
#4874=CARTESIAN_POINT ( 'NONE',  ( -11.24999999999996270, 12.50000000000000000, 6.560283801567334372 ) ) ;
#4875=DIRECTION ( 'NONE',  ( -0.000000000000000000, -1.000000000000000000, -0.000000000000000000 ) ) ;
#4876=DIRECTION ( 'NONE',  ( 0.000000000000000000, 0.000000000000000000, 1.000000000000000000 ) ) ;
#4877=AXIS2_PLACEMENT_3D ( 'NONE', #2511, #121656, #51654 ) ;
#4878=VERTEX_POINT ( 'NONE', #33795 ) ;
#4879=DIRECTION ( 'NONE',  ( 0.000000000000000000, 1.000000000000000000, 0.000000000000000000 ) ) ;
#4880=CIRCLE ( 'NONE', #32020, 0.06509327318403745899 ) ;
#4881=ADVANCED_FACE ( 'NONE', ( #113648 ), #11466, .T. ) ;
#4882=VECTOR ( 'NONE', #38306, 1000.000000000000000 ) ;
#4883=EDGE_LOOP ( 'NONE', ( #106955, #41863 ) ) ;
#4884=DIRECTION ( 'NONE',  ( -0.000000000000000000, 1.000000000000000000, -0.000000000000000000 ) ) ;
#4885=ORIENTED_EDGE ( 'NONE', *, *, #105281, .T. ) ;
#4886=DIRECTION ( 'NONE',  ( -0.000000000000000000, 1.000000000000000000, -0.000000000000000000 ) ) ;
#4888=CARTESIAN_POINT ( 'NONE',  ( 2.499999999999981792, 2.500000000000000000, 4.230127018922196669 ) ) ;
#4892=EDGE_CURVE ( 'NONE', #26341, #110101, #21861, .T. ) ;
#4893=ORIENTED_EDGE ( 'NONE', *, *, #19383, .F. ) ;
#4894=DIRECTION ( 'NONE',  ( 0.000000000000000000, 0.000000000000000000, -1.000000000000000000 ) ) ;
#4895=AXIS2_PLACEMENT_3D ( 'NONE', #21696, #4582, #72091 ) ;
#4896=EDGE_CURVE ( 'NONE', #87803, #2505, #80434, .T. ) ;
#4897=CARTESIAN_POINT ( 'NONE',  ( -6.450000000000019718, 12.50000000000000000, -6.148780366869526226 ) ) ;
#4898=ORIENTED_EDGE ( 'NONE', *, *, #74468, .T. ) ;
#4899=ORIENTED_EDGE ( 'NONE', *, *, #29341, .F. ) ;
#4900=ORIENTED_EDGE ( 'NONE', *, *, #63743, .T. ) ;
#4901=LINE ( 'NONE', #46132, #16523 ) ;
#4902=DIRECTION ( 'NONE',  ( 0.000000000000000000, 0.000000000000000000, 1.000000000000000000 ) ) ;
#4903=ADVANCED_FACE ( 'NONE', ( #48135 ), #17353, .T. ) ;
#4905=VECTOR ( 'NONE', #76346, 1000.000000000000000 ) ;
#4906=LINE ( 'NONE', #46793, #51308 ) ;
#4907=DIRECTION ( 'NONE',  ( 0.000000000000000000, -0.9999939076577903929, 0.003490651415223739937 ) ) ;
#4908=AXIS2_PLACEMENT_3D ( 'NONE', #31072, #70972, #21893 ) ;
#4909=CIRCLE ( 'NONE', #119851, 0.06509327318403741736 ) ;
#4910=AXIS2_PLACEMENT_3D ( 'NONE', #87452, #78312, #107751 ) ;
#4911=CARTESIAN_POINT ( 'NONE',  ( 0.000000000000000000, 2.500000000000000000, 0.1000000000000000056 ) ) ;
#4912=VECTOR ( 'NONE', #101764, 1000.000000000000000 ) ;
#4913=VERTEX_POINT ( 'NONE', #47491 ) ;
#4914=AXIS2_PLACEMENT_3D ( 'NONE', #122663, #80820, #102390 ) ;
#4915=DIRECTION ( 'NONE',  ( -0.000000000000000000, 1.000000000000000000, -0.000000000000000000 ) ) ;
#4916=ORIENTED_EDGE ( 'NONE', *, *, #51941, .T. ) ;
#4917=PLANE ( 'NONE',  #28498 ) ;
#4918=CARTESIAN_POINT ( 'NONE',  ( 4.149999999999938183, 12.50000000000000000, 7.188010851410848723 ) ) ;
#4919=FACE_OUTER_BOUND ( 'NONE', #69320, .T. ) ;
#4920=ORIENTED_EDGE ( 'NONE', *, *, #38781, .F. ) ;
#4921=DIRECTION ( 'NONE',  ( 0.000000000000000000, 0.000000000000000000, -1.000000000000000000 ) ) ;
#4923=CONICAL_SURFACE ( 'NONE', #84465, 0.1000000000000002554, 0.003490658503988666988 ) ;
#4924=ORIENTED_EDGE ( 'NONE', *, *, #8203, .F. ) ;
#4925=DIRECTION ( 'NONE',  ( 0.000000000000000000, -0.9999939076577903929, 0.003490651415223739937 ) ) ;
#4926=AXIS2_PLACEMENT_3D ( 'NONE', #66444, #67062, #107000 ) ;
#4927=ORIENTED_EDGE ( 'NONE', *, *, #66993, .T. ) ;
#4928=VECTOR ( 'NONE', #90141, 1000.000000000000000 ) ;
#4929=EDGE_LOOP ( 'NONE', ( #11971, #67160, #14044, #4195 ) ) ;
#4930=FACE_OUTER_BOUND ( 'NONE', #121558, .T. ) ;
#4931=CIRCLE ( 'NONE', #44678, 0.1000000000000000472 ) ;
#4932=AXIS2_PLACEMENT_3D ( 'NONE', #65610, #113427, #56429 ) ;
#4933=EDGE_CURVE ( 'NONE', #21022, #42779, #48782, .T. ) ;
#4935=ORIENTED_EDGE ( 'NONE', *, *, #60109, .T. ) ;
#4936=LINE ( 'NONE', #84800, #7019 ) ;
#4937=DIRECTION ( 'NONE',  ( 0.000000000000000000, 0.000000000000000000, 1.000000000000000000 ) ) ;
#4938=EDGE_CURVE ( 'NONE', #58767, #28931, #23992, .T. ) ;
#4939=FACE_OUTER_BOUND ( 'NONE', #128868, .T. ) ;
#4940=CONICAL_SURFACE ( 'NONE', #80183, 0.1000000000000002554, 0.003490658503988666988 ) ;
#4941=VERTEX_POINT ( 'NONE', #57308 ) ;
#4942=AXIS2_PLACEMENT_3D ( 'NONE', #33131, #121478, #61292 ) ;
#4943=CONICAL_SURFACE ( 'NONE', #90640, 0.09999999999999999167, 0.003490658503988666988 ) ;
#4944=FACE_BOUND ( 'NONE', #111556, .T. ) ;
#4945=EDGE_CURVE ( 'NONE', #34926, #65177, #63707, .T. ) ;
#4946=CARTESIAN_POINT ( 'NONE',  ( 11.24999999999991118, 2.500000000000000000, 5.802370205355744659 ) ) ;
#4947=CARTESIAN_POINT ( 'NONE',  ( -5.000000000000024869, 12.50000000000000000, -4.957854068765716882 ) ) ;
#4948=EDGE_LOOP ( 'NONE', ( #46157, #78105, #64882, #57992 ) ) ;
#4949=CONICAL_SURFACE ( 'NONE', #46838, 0.09999999999999982514, 0.003490658503988666988 ) ;
#4951=DIRECTION ( 'NONE',  ( 0.000000000000000000, 0.000000000000000000, 1.000000000000000000 ) ) ;
#4952=ORIENTED_EDGE ( 'NONE', *, *, #82872, .T. ) ;
#4953=EDGE_CURVE ( 'NONE', #9679, #29270, #101363, .T. ) ;
#4954=EDGE_CURVE ( 'NONE', #28355, #2437, #126393, .T. ) ;
#4955=VERTEX_POINT ( 'NONE', #7543 ) ;
#4956=VERTEX_POINT ( 'NONE', #88020 ) ;
#4957=DIRECTION ( 'NONE',  ( 0.000000000000000000, 0.000000000000000000, -1.000000000000000000 ) ) ;
#4958=DIRECTION ( 'NONE',  ( 0.000000000000000000, 0.000000000000000000, -1.000000000000000000 ) ) ;
#4959=FACE_OUTER_BOUND ( 'NONE', #90951, .T. ) ;
#4960=FACE_BOUND ( 'NONE', #56700, .T. ) ;
#4961=EDGE_LOOP ( 'NONE', ( #83025, #126071 ) ) ;
#4963=ADVANCED_FACE ( 'NONE', ( #98496 ), #13508, .T. ) ;
#4964=DIRECTION ( 'NONE',  ( -0.000000000000000000, 1.000000000000000000, -0.000000000000000000 ) ) ;
#4966=CONICAL_SURFACE ( 'NONE', #38449, 0.1000000000000002554, 0.003490658503988666988 ) ;
#4967=FACE_OUTER_BOUND ( 'NONE', #61566, .T. ) ;
#4968=DIRECTION ( 'NONE',  ( 0.000000000000000000, 0.000000000000000000, 1.000000000000000000 ) ) ;
#4969=FACE_OUTER_BOUND ( 'NONE', #36693, .T. ) ;
#4970=FACE_OUTER_BOUND ( 'NONE', #33727, .T. ) ;
#4971=AXIS2_PLACEMENT_3D ( 'NONE', #16198, #96064, #76434 ) ;
#4972=AXIS2_PLACEMENT_3D ( 'NONE', #41402, #2084, #102243 ) ;
#4973=AXIS2_PLACEMENT_3D ( 'NONE', #36707, #27487, #37975 ) ;
#4974=DIRECTION ( 'NONE',  ( 0.000000000000000000, -0.9999939076577903929, 0.003490651415223739937 ) ) ;
#4975=ORIENTED_EDGE ( 'NONE', *, *, #26952, .F. ) ;
#4976=ORIENTED_EDGE ( 'NONE', *, *, #21229, .T. ) ;
#4977=ORIENTED_EDGE ( 'NONE', *, *, #54533, .T. ) ;
#4978=ORIENTED_EDGE ( 'NONE', *, *, #121702, .T. ) ;
#4979=ORIENTED_EDGE ( 'NONE', *, *, #113099, .T. ) ;
#4980=CARTESIAN_POINT ( 'NONE',  ( -11.69999999999999929, 12.50000000000000000, -4.330127018922198978 ) ) ;
#4981=CARTESIAN_POINT ( 'NONE',  ( 6.249999999999968914, 2.500000000000000000, -6.395190528383301931 ) ) ;
#4982=VERTEX_POINT ( 'NONE', #8826 ) ;
#4983=FACE_BOUND ( 'NONE', #60629, .T. ) ;
#4984=CIRCLE ( 'NONE', #128357, 0.9999999999999995559 ) ;
#4985=DIRECTION ( 'NONE',  ( -4.274815082592931898E-19, -0.9999939076577903929, -0.003490651415223739937 ) ) ;
#4986=CIRCLE ( 'NONE', #63504, 0.1000000000000002554 ) ;
#4987=AXIS2_PLACEMENT_3D ( 'NONE', #93336, #82883, #122793 ) ;
#4988=FACE_OUTER_BOUND ( 'NONE', #27342, .T. ) ;
#4990=CARTESIAN_POINT ( 'NONE',  ( 1.049999999999953637, 2.500000000000000000, 2.511473670974873507 ) ) ;
#4991=DIRECTION ( 'NONE',  ( 0.000000000000000000, 1.000000000000000000, 0.000000000000000000 ) ) ;
#4992=DIRECTION ( 'NONE',  ( 0.000000000000000000, 0.000000000000000000, -1.000000000000000000 ) ) ;
#4993=AXIS2_PLACEMENT_3D ( 'NONE', #128017, #8232, #70389 ) ;
#4994=ORIENTED_EDGE ( 'NONE', *, *, #26972, .T. ) ;
#4995=DIRECTION ( 'NONE',  ( 0.000000000000000000, -0.9999939076577903929, 0.003490651415223739937 ) ) ;
#4996=EDGE_LOOP ( 'NONE', ( #23252, #114972 ) ) ;
#4997=EDGE_CURVE ( 'NONE', #108909, #47117, #97866, .T. ) ;
#4998=AXIS2_PLACEMENT_3D ( 'NONE', #119920, #87222, #127179 ) ;
#4999=CONICAL_SURFACE ( 'NONE', #109478, 0.09999999999999982514, 0.003490658503988666988 ) ;
#5000=AXIS2_PLACEMENT_3D ( 'NONE', #128475, #87863, #7377 ) ;
#5001=ORIENTED_EDGE ( 'NONE', *, *, #70586, .F. ) ;
#5002=EDGE_LOOP ( 'NONE', ( #33042, #3095 ) ) ;
#5003=CARTESIAN_POINT ( 'NONE',  ( 4.149999999999941735, 2.500000000000000000, -5.802370205355749988 ) ) ;
#5004=CARTESIAN_POINT ( 'NONE',  ( 6.249999999999932498, 2.500000000000000000, -5.902370205355750521 ) ) ;
#5005=DIRECTION ( 'NONE',  ( -4.274815082592931898E-19, -0.9999939076577903929, -0.003490651415223739937 ) ) ;
#5006=CIRCLE ( 'NONE', #65651, 0.1000000000000002554 ) ;
#5007=ORIENTED_EDGE ( 'NONE', *, *, #103438, .F. ) ;
#5008=CARTESIAN_POINT ( 'NONE',  ( 8.497934422630084583, 2.499999999999237499, -9.526046681105988512 ) ) ;
#5009=CIRCLE ( 'NONE', #128386, 0.09999999999999982514 ) ;
#5010=CARTESIAN_POINT ( 'NONE',  ( -8.350000000000013856, 2.500000000000000000, -6.495190528383297135 ) ) ;
#5011=CARTESIAN_POINT ( 'NONE',  ( -0.8500000000000386136, 2.500000000000000000, 5.802370205355744659 ) ) ;
#5013=DIRECTION ( 'NONE',  ( 0.000000000000000000, 0.000000000000000000, -1.000000000000000000 ) ) ;
#5014=CARTESIAN_POINT ( 'NONE',  ( 6.649999999999931077, 2.500000000000000000, -6.495190528383302464 ) ) ;
#5015=ORIENTED_EDGE ( 'NONE', *, *, #117211, .T. ) ;
#5016=CARTESIAN_POINT ( 'NONE',  ( -11.64999999999999680, 2.500000000000000000, -6.495190528383298911 ) ) ;
#5018=ORIENTED_EDGE ( 'NONE', *, *, #11367, .T. ) ;
#5019=DIRECTION ( 'NONE',  ( -0.000000000000000000, 1.000000000000000000, -0.000000000000000000 ) ) ;
#5020=FACE_OUTER_BOUND ( 'NONE', #35499, .T. ) ;
#5021=CIRCLE ( 'NONE', #120061, 0.06509327318403745899 ) ;
#5022=VECTOR ( 'NONE', #46939, 1000.000000000000000 ) ;
#5023=DIRECTION ( 'NONE',  ( -0.000000000000000000, 1.000000000000000000, -0.000000000000000000 ) ) ;
#5024=VECTOR ( 'NONE', #108530, 1000.000000000000000 ) ;
#5025=PLANE ( 'NONE',  #71779 ) ;
#5026=CARTESIAN_POINT ( 'NONE',  ( -3.750000000000027534, 2.500000000000000000, -1.572243186433550211 ) ) ;
#5027=VERTEX_POINT ( 'NONE', #128654 ) ;
#5028=VERTEX_POINT ( 'NONE', #126697 ) ;
#5029=CARTESIAN_POINT ( 'NONE',  ( 10.39999999999991154, 12.50000000000000000, -5.022947341949754119 ) ) ;
#5030=CONICAL_SURFACE ( 'NONE', #61500, 0.09999999999999982514, 0.003490658503988666988 ) ;
#5031=AXIS2_PLACEMENT_3D ( 'NONE', #117433, #19250, #38274 ) ;
#5032=CARTESIAN_POINT ( 'NONE',  ( 59.86262955839788447, 3.775832727647709497, -4.995375241584474324 ) ) ;
#5033=CIRCLE ( 'NONE', #107454, 0.1000000000000002554 ) ;
#5034=DIRECTION ( 'NONE',  ( 0.000000000000000000, 1.000000000000000000, 0.000000000000000000 ) ) ;
#5035=ORIENTED_EDGE ( 'NONE', *, *, #30435, .T. ) ;
#5036=VERTEX_POINT ( 'NONE', #67764 ) ;
#5037=LINE ( 'NONE', #94715, #114697 ) ;
#5038=ADVANCED_FACE ( 'NONE', ( #38989 ), #69968, .T. ) ;
#5040=CARTESIAN_POINT ( 'NONE',  ( -3.350000000000032507, 2.500000000000000000, -6.595190528383302109 ) ) ;
#5041=VECTOR ( 'NONE', #98844, 1000.000000000000000 ) ;
#5042=EDGE_CURVE ( 'NONE', #68393, #45115, #86679, .T. ) ;
#5043=DIRECTION ( 'NONE',  ( 0.000000000000000000, 0.000000000000000000, 1.000000000000000000 ) ) ;
#5044=ORIENTED_EDGE ( 'NONE', *, *, #46268, .T. ) ;
#5045=LINE ( 'NONE', #54169, #119264 ) ;
#5046=CARTESIAN_POINT ( 'NONE',  ( 0.5999999999999612310, 12.50000000000000000, -0.3464101615137760715 ) ) ;
#5047=CARTESIAN_POINT ( 'NONE',  ( 11.44999999999990870, 12.50000000000000000, 6.841600689897072485 ) ) ;
#5048=CONICAL_SURFACE ( 'NONE', #74016, 0.1000000000000002554, 0.003490658503988666988 ) ;
#5049=EDGE_CURVE ( 'NONE', #23957, #55213, #103415, .T. ) ;
#5050=DIRECTION ( 'NONE',  ( -0.000000000000000000, -1.000000000000000000, -0.000000000000000000 ) ) ;
#5051=EDGE_CURVE ( 'NONE', #58166, #52632, #113880, .T. ) ;
#5052=ORIENTED_EDGE ( 'NONE', *, *, #108774, .T. ) ;
#5053=CARTESIAN_POINT ( 'NONE',  ( -12.29999999999999361, 2.500000000000000000, 3.883716857408420431 ) ) ;
#5055=EDGE_CURVE ( 'NONE', #92856, #126533, #1005, .T. ) ;
#5056=ORIENTED_EDGE ( 'NONE', *, *, #91059, .F. ) ;
#5057=EDGE_CURVE ( 'NONE', #63382, #73184, #36528, .T. ) ;
#5059=ORIENTED_EDGE ( 'NONE', *, *, #24741, .T. ) ;
#5060=EDGE_CURVE ( 'NONE', #15503, #19409, #74169, .T. ) ;
#5062=DIRECTION ( 'NONE',  ( 0.000000000000000000, -0.000000000000000000, 1.000000000000000000 ) ) ;
#5063=EDGE_CURVE ( 'NONE', #93363, #81045, #10746, .T. ) ;
#5064=EDGE_CURVE ( 'NONE', #41827, #90531, #76230, .T. ) ;
#5065=DIRECTION ( 'NONE',  ( 0.000000000000000000, 0.000000000000000000, 1.000000000000000000 ) ) ;
#5066=CIRCLE ( 'NONE', #78251, 0.06509327318403745899 ) ;
#5067=LINE ( 'NONE', #125490, #122120 ) ;
#5068=CARTESIAN_POINT ( 'NONE',  ( -3.550000000000027356, 12.50000000000000000, -2.511473670974877948 ) ) ;
#5069=CARTESIAN_POINT ( 'NONE',  ( 15.83209681635554666, 2.500000000000000000, -5.404881881984140435 ) ) ;
#5070=DIRECTION ( 'NONE',  ( 0.000000000000000000, 0.000000000000000000, -1.000000000000000000 ) ) ;
#5072=DIRECTION ( 'NONE',  ( -0.000000000000000000, 1.000000000000000000, -0.000000000000000000 ) ) ;
#5073=EDGE_CURVE ( 'NONE', #72972, #97694, #109677, .T. ) ;
#5074=DIRECTION ( 'NONE',  ( -0.000000000000000000, -1.000000000000000000, -0.000000000000000000 ) ) ;
#5075=VERTEX_POINT ( 'NONE', #22553 ) ;
#5076=CIRCLE ( 'NONE', #109554, 0.1000000000000002554 ) ;
#5077=EDGE_LOOP ( 'NONE', ( #70411, #17156, #19043, #78322 ) ) ;
#5078=VERTEX_POINT ( 'NONE', #23166 ) ;
#5079=ORIENTED_EDGE ( 'NONE', *, *, #117055, .F. ) ;
#5080=DIRECTION ( 'NONE',  ( 0.000000000000000000, 0.000000000000000000, -1.000000000000000000 ) ) ;
#5081=DIRECTION ( 'NONE',  ( 0.000000000000000000, 0.000000000000000000, 1.000000000000000000 ) ) ;
#5082=CARTESIAN_POINT ( 'NONE',  ( 4.349999999999937472, 2.500000000000000000, 6.741600689897071952 ) ) ;
#5083=ORIENTED_EDGE ( 'NONE', *, *, #121374, .F. ) ;
#5084=DIRECTION ( 'NONE',  ( 0.000000000000000000, 1.000000000000000000, 0.000000000000000000 ) ) ;
#5085=CIRCLE ( 'NONE', #117952, 0.1000000000000000472 ) ;
#5086=CARTESIAN_POINT ( 'NONE',  ( -7.050000000000016698, 2.500000000000000000, -6.495190528383302464 ) ) ;
#5087=FACE_OUTER_BOUND ( 'NONE', #58025, .T. ) ;
#5088=ORIENTED_EDGE ( 'NONE', *, *, #7587, .T. ) ;
#5089=CARTESIAN_POINT ( 'NONE',  ( 1.049999999999954081, 2.500000000000000000, -6.148780366869526226 ) ) ;
#5090=VERTEX_POINT ( 'NONE', #21905 ) ;
#5091=AXIS2_PLACEMENT_3D ( 'NONE', #62301, #102220, #32847 ) ;
#5092=VECTOR ( 'NONE', #126057, 1000.000000000000000 ) ;
#5093=ORIENTED_EDGE ( 'NONE', *, *, #5228, .T. ) ;
#5094=VERTEX_POINT ( 'NONE', #52004 ) ;
#5095=ORIENTED_EDGE ( 'NONE', *, *, #86730, .T. ) ;
#5096=CARTESIAN_POINT ( 'NONE',  ( -0.8500000000000390576, 12.50000000000000000, -2.099970236277064473 ) ) ;
#5097=CIRCLE ( 'NONE', #90788, 0.1000000000000000472 ) ;
#5098=EDGE_CURVE ( 'NONE', #37944, #84568, #95005, .T. ) ;
#5099=FACE_OUTER_BOUND ( 'NONE', #17057, .T. ) ;
#5100=DIRECTION ( 'NONE',  ( 0.000000000000000000, 1.000000000000000000, 0.000000000000000000 ) ) ;
#5101=EDGE_CURVE ( 'NONE', #3892, #26528, #49052, .T. ) ;
#5102=CONICAL_SURFACE ( 'NONE', #53246, 0.1000000000000000472, 0.003490658503988666988 ) ;
#5103=FACE_OUTER_BOUND ( 'NONE', #88549, .T. ) ;
#5104=ORIENTED_EDGE ( 'NONE', *, *, #67744, .F. ) ;
#5105=EDGE_CURVE ( 'NONE', #111372, #122281, #21957, .T. ) ;
#5106=DIRECTION ( 'NONE',  ( -0.000000000000000000, -1.000000000000000000, -0.000000000000000000 ) ) ;
#5107=ORIENTED_EDGE ( 'NONE', *, *, #111762, .T. ) ;
#5108=LINE ( 'NONE', #26055, #78958 ) ;
#5110=DIRECTION ( 'NONE',  ( 0.000000000000000000, 0.000000000000000000, 1.000000000000000000 ) ) ;
#5111=CARTESIAN_POINT ( 'NONE',  ( 16.09541403888747624, -2.463474929527651458, 3.723514363708886776 ) ) ;
#5112=EDGE_CURVE ( 'NONE', #120069, #17444, #15651, .T. ) ;
#5113=EDGE_CURVE ( 'NONE', #114788, #10245, #78383, .T. ) ;
#5114=ORIENTED_EDGE ( 'NONE', *, *, #22390, .T. ) ;
#5115=ADVANCED_FACE ( 'NONE', ( #50700 ), #110898, .T. ) ;
#5116=EDGE_CURVE ( 'NONE', #49994, #107746, #95099, .T. ) ;
#5117=VECTOR ( 'NONE', #81844, 1000.000000000000000 ) ;
#5118=VERTEX_POINT ( 'NONE', #111554 ) ;
#5119=ORIENTED_EDGE ( 'NONE', *, *, #24766, .F. ) ;
#5120=CARTESIAN_POINT ( 'NONE',  ( -4.600000000000024514, 12.50000000000000000, 0.6928203230275494784 ) ) ;
#5121=FACE_OUTER_BOUND ( 'NONE', #119665, .T. ) ;
#5122=DIRECTION ( 'NONE',  ( 0.000000000000000000, 0.000000000000000000, 1.000000000000000000 ) ) ;
#5123=FACE_BOUND ( 'NONE', #122538, .T. ) ;
#5124=CARTESIAN_POINT ( 'NONE',  ( -6.650000000000019007, 12.50000000000000000, -1.472243186433550122 ) ) ;
#5125=DIRECTION ( 'NONE',  ( 0.000000000000000000, 0.000000000000000000, 1.000000000000000000 ) ) ;
#5126=EDGE_CURVE ( 'NONE', #91178, #77609, #32432, .T. ) ;
#5127=CARTESIAN_POINT ( 'NONE',  ( -4.600000000000024514, 2.500000000000000000, 0.5928203230275495006 ) ) ;
#5128=CIRCLE ( 'NONE', #19813, 0.06509327318403745899 ) ;
#5129=VECTOR ( 'NONE', #55090, 1000.000000000000000 ) ;
#5130=VECTOR ( 'NONE', #23788, 1000.000000000000000 ) ;
#5131=CARTESIAN_POINT ( 'NONE',  ( -2.900000000000029221, 12.50000000000000000, -0.6277270498435166823 ) ) ;
#5132=VECTOR ( 'NONE', #119709, 1000.000000000000000 ) ;
#5133=CARTESIAN_POINT ( 'NONE',  ( 5.399999999999931966, 12.50000000000000000, 4.265033745738159077 ) ) ;
#5134=FACE_OUTER_BOUND ( 'NONE', #43130, .T. ) ;
#5135=ORIENTED_EDGE ( 'NONE', *, *, #12320, .F. ) ;
#5136=VECTOR ( 'NONE', #127583, 1000.000000000000000 ) ;
#5137=CIRCLE ( 'NONE', #120082, 0.1000000000000000472 ) ;
#5138=CARTESIAN_POINT ( 'NONE',  ( 3.149999999999946176, 2.500000000000000000, -6.741600689897077281 ) ) ;
#5139=ORIENTED_EDGE ( 'NONE', *, *, #105703, .F. ) ;
#5140=EDGE_LOOP ( 'NONE', ( #95781, #109775, #28832, #97676 ) ) ;
#5141=VERTEX_POINT ( 'NONE', #40915 ) ;
#5142=EDGE_LOOP ( 'NONE', ( #74538, #112223, #95546, #125646 ) ) ;
#5143=AXIS2_PLACEMENT_3D ( 'NONE', #93465, #13598, #14866 ) ;
#5144=CARTESIAN_POINT ( 'NONE',  ( -2.050000000000033129, 2.500000000000000000, 2.265063509461097357 ) ) ;
#5145=EDGE_CURVE ( 'NONE', #53201, #5697, #61170, .T. ) ;
#5146=FACE_BOUND ( 'NONE', #2391, .T. ) ;
#5148=ORIENTED_EDGE ( 'NONE', *, *, #112779, .F. ) ;
#5149=CARTESIAN_POINT ( 'NONE',  ( 24.00496409367085704, 0.9037364216963271746, 4.313973893093799639 ) ) ;
#5150=FACE_OUTER_BOUND ( 'NONE', #95012, .T. ) ;
#5151=VECTOR ( 'NONE', #69136, 1000.000000000000000 ) ;
#5152=VERTEX_POINT ( 'NONE', #92559 ) ;
#5153=DIRECTION ( 'NONE',  ( 0.000000000000000000, -0.000000000000000000, 1.000000000000000000 ) ) ;
#5154=DIRECTION ( 'NONE',  ( 0.000000000000000000, 0.000000000000000000, -1.000000000000000000 ) ) ;
#5155=ADVANCED_FACE ( 'NONE', ( #112207 ), #62477, .T. ) ;
#5156=ORIENTED_EDGE ( 'NONE', *, *, #94770, .F. ) ;
#5157=DIRECTION ( 'NONE',  ( 0.000000000000000000, 0.000000000000000000, 1.000000000000000000 ) ) ;
#5159=AXIS2_PLACEMENT_3D ( 'NONE', #24010, #72471, #62655 ) ;
#5160=AXIS2_PLACEMENT_3D ( 'NONE', #26721, #55542, #105926 ) ;
#5161=ORIENTED_EDGE ( 'NONE', *, *, #48364, .T. ) ;
#5162=DIRECTION ( 'NONE',  ( -0.000000000000000000, -1.000000000000000000, -0.000000000000000000 ) ) ;
#5163=CARTESIAN_POINT ( 'NONE',  ( 12.29999999999990479, 12.50000000000000000, 4.676537180435972552 ) ) ;
#5164=ORIENTED_EDGE ( 'NONE', *, *, #4452, .F. ) ;
#5165=ORIENTED_EDGE ( 'NONE', *, *, #4306, .T. ) ;
#5166=ADVANCED_FACE ( 'NONE', ( #52630 ), #33020, .T. ) ;
#5167=DIRECTION ( 'NONE',  ( 0.000000000000000000, 0.000000000000000000, 1.000000000000000000 ) ) ;
#5168=VERTEX_POINT ( 'NONE', #54551 ) ;
#5169=CARTESIAN_POINT ( 'NONE',  ( 17.50000000000000000, -2.500000000000000000, -2.922290670087884124 ) ) ;
#5170=DIRECTION ( 'NONE',  ( 0.000000000000000000, 0.000000000000000000, 1.000000000000000000 ) ) ;
#5171=CIRCLE ( 'NONE', #78365, 0.1000000000000002554 ) ;
#5172=ORIENTED_EDGE ( 'NONE', *, *, #81372, .T. ) ;
#5173=CARTESIAN_POINT ( 'NONE',  ( -6.250000000000021316, 12.50000000000000000, -5.802370205355749988 ) ) ;
#5174=DIRECTION ( 'NONE',  ( -0.000000000000000000, 1.000000000000000000, -0.000000000000000000 ) ) ;
#5175=LINE ( 'NONE', #45127, #46627 ) ;
#5176=FACE_OUTER_BOUND ( 'NONE', #48615, .T. ) ;
#5177=DIRECTION ( 'NONE',  ( 0.000000000000000000, 0.000000000000000000, -1.000000000000000000 ) ) ;
#5178=EDGE_LOOP ( 'NONE', ( #95951, #113524 ) ) ;
#5179=ORIENTED_EDGE ( 'NONE', *, *, #23707, .F. ) ;
#5180=FACE_OUTER_BOUND ( 'NONE', #117236, .T. ) ;
#5181=AXIS2_PLACEMENT_3D ( 'NONE', #62153, #625, #80504 ) ;
#5182=CONICAL_SURFACE ( 'NONE', #128571, 0.1000000000000002554, 0.003490658503988666988 ) ;
#5183=DIRECTION ( 'NONE',  ( -0.000000000000000000, -1.000000000000000000, -0.000000000000000000 ) ) ;
#5184=CARTESIAN_POINT ( 'NONE',  ( 11.44999999999990514, 2.500000000000000000, -6.048780366869526581 ) ) ;
#5185=ORIENTED_EDGE ( 'NONE', *, *, #14288, .F. ) ;
#5186=ORIENTED_EDGE ( 'NONE', *, *, #51232, .F. ) ;
#5187=EDGE_LOOP ( 'NONE', ( #48315, #57710 ) ) ;
#5188=CIRCLE ( 'NONE', #90885, 0.09999999999999982514 ) ;
#5189=CARTESIAN_POINT ( 'NONE',  ( 2.899999999999946620, 2.500000000000000000, 0.6928203230275494784 ) ) ;
#5190=AXIS2_PLACEMENT_3D ( 'NONE', #112853, #60552, #12061 ) ;
#5191=DIRECTION ( 'NONE',  ( 0.000000000000000000, 0.000000000000000000, 1.000000000000000000 ) ) ;
#5192=CARTESIAN_POINT ( 'NONE',  ( -8.300000000000011369, 2.500000000000000000, -4.430127018922202176 ) ) ;
#5193=EDGE_CURVE ( 'NONE', #4124, #949, #119951, .T. ) ;
#5195=CARTESIAN_POINT ( 'NONE',  ( -3.950000000000024603, 2.500000000000000000, 1.918653347947321564 ) ) ;
#5197=DIRECTION ( 'NONE',  ( 0.000000000000000000, 0.000000000000000000, -1.000000000000000000 ) ) ;
#5198=FACE_OUTER_BOUND ( 'NONE', #122937, .T. ) ;
#5199=PLANE ( 'NONE',  #63437 ) ;
#5200=CARTESIAN_POINT ( 'NONE',  ( -0.2000000000000412836, 2.500000000000000000, 4.676537180435972552 ) ) ;
#5201=EDGE_LOOP ( 'NONE', ( #55497, #48337 ) ) ;
#5202=AXIS2_PLACEMENT_3D ( 'NONE', #78510, #25497, #5859 ) ;
#5203=VECTOR ( 'NONE', #100538, 1000.000000000000000 ) ;
#5204=CARTESIAN_POINT ( 'NONE',  ( -2.950000000000029932, 2.500000000000000000, -2.165063509461101710 ) ) ;
#5205=EDGE_CURVE ( 'NONE', #42741, #60040, #122013, .T. ) ;
#5206=AXIS2_PLACEMENT_3D ( 'NONE', #34509, #84870, #63298 ) ;
#5207=ORIENTED_EDGE ( 'NONE', *, *, #12039, .T. ) ;
#5208=EDGE_CURVE ( 'NONE', #82898, #110307, #74214, .T. ) ;
#5209=ORIENTED_EDGE ( 'NONE', *, *, #55722, .T. ) ;
#5210=EDGE_CURVE ( 'NONE', #59339, #123245, #34290, .T. ) ;
#5211=DIRECTION ( 'NONE',  ( 0.000000000000000000, 1.000000000000000000, 0.000000000000000000 ) ) ;
#5212=CARTESIAN_POINT ( 'NONE',  ( -12.49999999999995737, 2.500000000000000000, 4.230127018922196669 ) ) ;
#5213=ADVANCED_FACE ( 'NONE', ( #34950 ), #84352, .T. ) ;
#5214=DIRECTION ( 'NONE',  ( 0.000000000000000000, -0.9999939076577903929, 0.003490651415223739937 ) ) ;
#5215=CIRCLE ( 'NONE', #105584, 0.06509327318403745899 ) ;
#5216=CARTESIAN_POINT ( 'NONE',  ( 12.49999999999990408, 2.500000000000000000, 4.922947341949748257 ) ) ;
#5217=AXIS2_PLACEMENT_3D ( 'NONE', #54285, #66668, #85673 ) ;
#5218=AXIS2_PLACEMENT_3D ( 'NONE', #80091, #31015, #32309 ) ;
#5219=DIRECTION ( 'NONE',  ( 0.000000000000000000, 0.000000000000000000, -1.000000000000000000 ) ) ;
#5220=ADVANCED_FACE ( 'NONE', ( #66314 ), #65569, .T. ) ;
#5221=FACE_OUTER_BOUND ( 'NONE', #89162, .T. ) ;
#5222=DIRECTION ( 'NONE',  ( -4.274815082592931898E-19, -0.9999939076577903929, -0.003490651415223739937 ) ) ;
#5223=VERTEX_POINT ( 'NONE', #114768 ) ;
#5224=DIRECTION ( 'NONE',  ( 0.000000000000000000, 1.000000000000000000, 0.000000000000000000 ) ) ;
#5225=AXIS2_PLACEMENT_3D ( 'NONE', #47612, #77065, #87509 ) ;
#5226=ADVANCED_FACE ( 'NONE', ( #33646 ), #80251, .T. ) ;
#5227=DIRECTION ( 'NONE',  ( -0.000000000000000000, 1.000000000000000000, -0.000000000000000000 ) ) ;
#5228=EDGE_CURVE ( 'NONE', #26496, #18441, #125246, .T. ) ;
#5229=CIRCLE ( 'NONE', #57477, 0.06509327318403745899 ) ;
#5230=EDGE_LOOP ( 'NONE', ( #47623, #1173 ) ) ;
#5231=AXIS2_PLACEMENT_3D ( 'NONE', #3562, #4830, #43506 ) ;
#5232=EDGE_CURVE ( 'NONE', #18500, #90643, #55115, .T. ) ;
#5233=VERTEX_POINT ( 'NONE', #44099 ) ;
#5234=EDGE_LOOP ( 'NONE', ( #57950, #100376 ) ) ;
#5235=CONICAL_SURFACE ( 'NONE', #103545, 0.09999999999999982514, 0.003490658503988666988 ) ;
#5237=ORIENTED_EDGE ( 'NONE', *, *, #17928, .F. ) ;
#5238=EDGE_CURVE ( 'NONE', #21571, #58472, #23813, .T. ) ;
#5239=DIRECTION ( 'NONE',  ( 0.000000000000000000, 0.000000000000000000, 1.000000000000000000 ) ) ;
#5240=DIRECTION ( 'NONE',  ( -0.000000000000000000, -1.000000000000000000, -0.000000000000000000 ) ) ;
#5241=CARTESIAN_POINT ( 'NONE',  ( 16.55763164795904174, -0.1615198509451942488, -6.093150836621332722 ) ) ;
#5242=CARTESIAN_POINT ( 'NONE',  ( -11.05000000000000071, 2.500000000000000000, -6.741600689897074616 ) ) ;
#5243=LINE ( 'NONE', #74634, #61788 ) ;
#5244=ORIENTED_EDGE ( 'NONE', *, *, #9392, .F. ) ;
#5245=CARTESIAN_POINT ( 'NONE',  ( 3.549999999999940314, 2.500000000000000000, 6.741600689897071952 ) ) ;
#5246=CARTESIAN_POINT ( 'NONE',  ( 7.949999999999922018, 12.50000000000000000, 6.495190528383297135 ) ) ;
#5247=AXIS2_PLACEMENT_3D ( 'NONE', #70212, #110764, #110132 ) ;
#5248=CARTESIAN_POINT ( 'NONE',  ( 1.849999999999949685, 2.500000000000000000, -2.411473670974877859 ) ) ;
#5249=ORIENTED_EDGE ( 'NONE', *, *, #93634, .F. ) ;
#5251=ORIENTED_EDGE ( 'NONE', *, *, #54967, .T. ) ;
#5252=CARTESIAN_POINT ( 'NONE',  ( -3.950000000000029932, 12.50000000000000000, -6.083687093685488989 ) ) ;
#5253=CIRCLE ( 'NONE', #53308, 0.1000000000000002554 ) ;
#5254=FACE_OUTER_BOUND ( 'NONE', #120150, .T. ) ;
#5255=FACE_OUTER_BOUND ( 'NONE', #26043, .T. ) ;
#5256=ORIENTED_EDGE ( 'NONE', *, *, #23355, .F. ) ;
#5257=CARTESIAN_POINT ( 'NONE',  ( 6.049999999999935874, 2.500000000000000000, -6.741600689897077281 ) ) ;
#5258=CARTESIAN_POINT ( 'NONE',  ( -8.150000000000012790, 12.50000000000000000, -1.818653347947326138 ) ) ;
#5259=CARTESIAN_POINT ( 'NONE',  ( -7.300000000000016698, 12.50000000000000000, -0.2813168883297409439 ) ) ;
#5261=LINE ( 'NONE', #13790, #72862 ) ;
#5262=CONICAL_SURFACE ( 'NONE', #78461, 0.1000000000000000472, 0.003490658503988666988 ) ;
#5263=EDGE_CURVE ( 'NONE', #112855, #38253, #105283, .T. ) ;
#5264=VERTEX_POINT ( 'NONE', #105612 ) ;
#5266=AXIS2_PLACEMENT_3D ( 'NONE', #24809, #94834, #5154 ) ;
#5267=ADVANCED_FACE ( 'NONE', ( #46050 ), #116060, .T. ) ;
#5268=EDGE_LOOP ( 'NONE', ( #98109, #36872 ) ) ;
#5269=EDGE_LOOP ( 'NONE', ( #112041, #86507, #20833, #10520 ) ) ;
#5271=CARTESIAN_POINT ( 'NONE',  ( 1.049999999999953637, 12.50000000000000000, 2.511473670974873507 ) ) ;
#5272=FACE_BOUND ( 'NONE', #17793, .T. ) ;
#5273=CARTESIAN_POINT ( 'NONE',  ( -1.250000000000035749, 2.500000000000000000, -2.857883832488653741 ) ) ;
#5274=EDGE_CURVE ( 'NONE', #104358, #12341, #51015, .T. ) ;
#5275=DIRECTION ( 'NONE',  ( -0.000000000000000000, 1.000000000000000000, -0.000000000000000000 ) ) ;
#5276=AXIS2_PLACEMENT_3D ( 'NONE', #64390, #51375, #91278 ) ;
#5277=CIRCLE ( 'NONE', #67977, 0.1000000000000002554 ) ;
#5278=ORIENTED_EDGE ( 'NONE', *, *, #23064, .F. ) ;
#5279=CARTESIAN_POINT ( 'NONE',  ( -14.99999999999994671, 2.500000000000000000, -0.1000000000000000056 ) ) ;
#5280=DIRECTION ( 'NONE',  ( 0.000000000000000000, 0.000000000000000000, 1.000000000000000000 ) ) ;
#5281=CARTESIAN_POINT ( 'NONE',  ( 11.04999999999990834, 12.50000000000000000, -6.906693963081115051 ) ) ;
#5282=DIRECTION ( 'NONE',  ( 0.000000000000000000, 0.000000000000000000, 1.000000000000000000 ) ) ;
#5283=EDGE_LOOP ( 'NONE', ( #93950, #81481 ) ) ;
#5284=CARTESIAN_POINT ( 'NONE',  ( -8.550000000000007816, 12.50000000000000000, 6.148780366869520009 ) ) ;
#5286=CIRCLE ( 'NONE', #59710, 0.1000000000000000056 ) ;
#5287=EDGE_LOOP ( 'NONE', ( #14898, #42890 ) ) ;
#5288=DIRECTION ( 'NONE',  ( -0.000000000000000000, 1.000000000000000000, -0.000000000000000000 ) ) ;
#5289=AXIS2_PLACEMENT_3D ( 'NONE', #128226, #18891, #68642 ) ;
#5290=EDGE_LOOP ( 'NONE', ( #124242, #93623, #55790, #42089 ) ) ;
#5291=FACE_BOUND ( 'NONE', #14517, .T. ) ;
#5292=DIRECTION ( 'NONE',  ( 0.000000000000000000, 0.000000000000000000, 1.000000000000000000 ) ) ;
#5293=CIRCLE ( 'NONE', #118177, 0.06509327318403745899 ) ;
#5294=ORIENTED_EDGE ( 'NONE', *, *, #41057, .T. ) ;
#5295=CARTESIAN_POINT ( 'NONE',  ( -6.850000000000017408, 12.50000000000000000, -6.083687093685488989 ) ) ;
#5296=DIRECTION ( 'NONE',  ( -0.000000000000000000, -1.000000000000000000, -0.000000000000000000 ) ) ;
#5297=AXIS2_PLACEMENT_3D ( 'NONE', #16014, #44193, #125344 ) ;
#5298=VECTOR ( 'NONE', #66199, 1000.000000000000000 ) ;
#5299=ORIENTED_EDGE ( 'NONE', *, *, #73497, .T. ) ;
#5300=ORIENTED_EDGE ( 'NONE', *, *, #58998, .F. ) ;
#5302=ORIENTED_EDGE ( 'NONE', *, *, #70127, .T. ) ;
#5303=CARTESIAN_POINT ( 'NONE',  ( -14.79999999999998472, 12.50000000000000000, 0.4115034346978132529 ) ) ;
#5304=DIRECTION ( 'NONE',  ( 0.000000000000000000, 1.000000000000000000, 0.000000000000000000 ) ) ;
#5305=AXIS2_PLACEMENT_3D ( 'NONE', #99376, #9696, #37863 ) ;
#5306=CIRCLE ( 'NONE', #120261, 0.09999999999999999167 ) ;
#5307=CARTESIAN_POINT ( 'NONE',  ( 12.09999999999990550, 2.500000000000000000, -4.230127018922201998 ) ) ;
#5308=CARTESIAN_POINT ( 'NONE',  ( -4.120979160187744630E-14, 12.50000000000000000, 3.572213422710607489 ) ) ;
#5309=AXIS2_PLACEMENT_3D ( 'NONE', #99289, #121479, #39094 ) ;
#5310=DIRECTION ( 'NONE',  ( -0.000000000000000000, -1.000000000000000000, -0.000000000000000000 ) ) ;
#5311=CARTESIAN_POINT ( 'NONE',  ( -4.600000000000025402, 2.500000000000000000, 0.09999999999999761857 ) ) ;
#5312=CIRCLE ( 'NONE', #122329, 0.06509327318403745899 ) ;
#5313=VECTOR ( 'NONE', #22428, 1000.000000000000000 ) ;
#5314=VERTEX_POINT ( 'NONE', #104938 ) ;
#5315=AXIS2_PLACEMENT_3D ( 'NONE', #11323, #100356, #99715 ) ;
#5316=VERTEX_POINT ( 'NONE', #55223 ) ;
#5317=CARTESIAN_POINT ( 'NONE',  ( 7.899999999999924860, 2.500000000000000000, -4.922947341949753586 ) ) ;
#5318=LINE ( 'NONE', #45265, #127083 ) ;
#5319=CARTESIAN_POINT ( 'NONE',  ( -2.500000000000032419, 12.50000000000000000, 0.6928203230275494784 ) ) ;
#5320=CONICAL_SURFACE ( 'NONE', #59739, 0.1000000000000000472, 0.003490658503988666988 ) ;
#5321=EDGE_CURVE ( 'NONE', #95827, #3051, #96958, .T. ) ;
#5322=CARTESIAN_POINT ( 'NONE',  ( -4.999999999999986677, 12.50000000000000000, -0.06509327318403970719 ) ) ;
#5323=ORIENTED_EDGE ( 'NONE', *, *, #19091, .T. ) ;
#5324=ORIENTED_EDGE ( 'NONE', *, *, #86536, .F. ) ;
#5325=CARTESIAN_POINT ( 'NONE',  ( -10.45000000000000462, 12.50000000000000000, -2.230156782645135394 ) ) ;
#5326=ORIENTED_EDGE ( 'NONE', *, *, #124740, .T. ) ;
#5327=ADVANCED_FACE ( 'NONE', ( #95783 ), #25865, .T. ) ;
#5328=FACE_OUTER_BOUND ( 'NONE', #22977, .T. ) ;
#5330=ORIENTED_EDGE ( 'NONE', *, *, #51787, .T. ) ;
#5331=CARTESIAN_POINT ( 'NONE',  ( -14.39999999999998614, 12.50000000000000000, -0.4115034346978134749 ) ) ;
#5332=CARTESIAN_POINT ( 'NONE',  ( -3.550000000000027356, 12.50000000000000000, 1.818653347947321475 ) ) ;
#5333=PLANE ( 'NONE',  #45106 ) ;
#5334=PLANE ( 'NONE',  #109273 ) ;
#5335=CARTESIAN_POINT ( 'NONE',  ( -8.750000000000010658, 2.500000000000000000, 2.957883832488649389 ) ) ;
#5336=CARTESIAN_POINT ( 'NONE',  ( 1.249999999999952038, 2.500000000000000000, 2.757883832488649656 ) ) ;
#5337=EDGE_CURVE ( 'NONE', #50344, #10471, #82309, .T. ) ;
#5339=DIRECTION ( 'NONE',  ( -0.000000000000000000, -1.000000000000000000, -0.000000000000000000 ) ) ;
#5340=AXIS2_PLACEMENT_3D ( 'NONE', #125727, #67438, #47198 ) ;
#5341=CARTESIAN_POINT ( 'NONE',  ( 13.34999999999990017, 2.500000000000000000, 1.472243186433545459 ) ) ;
#5342=ORIENTED_EDGE ( 'NONE', *, *, #125933, .F. ) ;
#5343=VERTEX_POINT ( 'NONE', #83400 ) ;
#5344=DIRECTION ( 'NONE',  ( 0.000000000000000000, -0.000000000000000000, 1.000000000000000000 ) ) ;
#5345=ORIENTED_EDGE ( 'NONE', *, *, #110778, .T. ) ;
#5346=DIRECTION ( 'NONE',  ( 0.000000000000000000, 0.000000000000000000, 1.000000000000000000 ) ) ;
#5347=ORIENTED_EDGE ( 'NONE', *, *, #99969, .T. ) ;
#5348=ORIENTED_EDGE ( 'NONE', *, *, #37774, .T. ) ;
#5349=AXIS2_PLACEMENT_3D ( 'NONE', #25606, #85184, #83268 ) ;
#5350=ORIENTED_EDGE ( 'NONE', *, *, #118188, .T. ) ;
#5351=DIRECTION ( 'NONE',  ( 0.000000000000000000, 0.000000000000000000, 1.000000000000000000 ) ) ;
#5352=CONICAL_SURFACE ( 'NONE', #1153, 0.1000000000000002554, 0.003490658503988666988 ) ;
#5353=AXIS2_PLACEMENT_3D ( 'NONE', #77578, #79537, #117485 ) ;
#5354=CARTESIAN_POINT ( 'NONE',  ( -14.34999999999998543, 2.500000000000000000, -1.818653347947323695 ) ) ;
#5355=EDGE_CURVE ( 'NONE', #109519, #64213, #8663, .T. ) ;
#5356=DIRECTION ( 'NONE',  ( 0.000000000000000000, 0.000000000000000000, 1.000000000000000000 ) ) ;
#5357=CARTESIAN_POINT ( 'NONE',  ( -10.65000000000000213, 2.500000000000000000, 2.411473670974873862 ) ) ;
#5359=ORIENTED_EDGE ( 'NONE', *, *, #13084, .T. ) ;
#5360=CARTESIAN_POINT ( 'NONE',  ( 11.44999999999990514, 12.50000000000000000, -6.213873640053564351 ) ) ;
#5361=ORIENTED_EDGE ( 'NONE', *, *, #43244, .T. ) ;
#5362=CONICAL_SURFACE ( 'NONE', #95265, 0.09999999999999982514, 0.003490658503988666988 ) ;
#5363=EDGE_CURVE ( 'NONE', #80231, #80146, #99005, .T. ) ;
#5364=ORIENTED_EDGE ( 'NONE', *, *, #19444, .F. ) ;
#5365=ORIENTED_EDGE ( 'NONE', *, *, #71201, .F. ) ;
#5366=CARTESIAN_POINT ( 'NONE',  ( 11.04999999999991189, 12.50000000000000000, -2.511473670974877948 ) ) ;
#5367=EDGE_CURVE ( 'NONE', #88198, #123035, #44652, .T. ) ;
#5368=ORIENTED_EDGE ( 'NONE', *, *, #19046, .T. ) ;
#5369=EDGE_CURVE ( 'NONE', #43040, #87465, #9334, .T. ) ;
#5370=VERTEX_POINT ( 'NONE', #7385 ) ;
#5371=EDGE_CURVE ( 'NONE', #128977, #114770, #40557, .T. ) ;
#5372=ORIENTED_EDGE ( 'NONE', *, *, #1955, .F. ) ;
#5373=EDGE_CURVE ( 'NONE', #16094, #48072, #88530, .T. ) ;
#5374=CARTESIAN_POINT ( 'NONE',  ( 11.24999999999990585, 2.500000000000000000, 2.857883832488649301 ) ) ;
#5375=DIRECTION ( 'NONE',  ( 0.000000000000000000, 0.000000000000000000, -1.000000000000000000 ) ) ;
#5376=CIRCLE ( 'NONE', #13684, 0.09999999999999982514 ) ;
#5377=CARTESIAN_POINT ( 'NONE',  ( -12.69999999999999218, 2.500000000000000000, -4.776537180435974861 ) ) ;
#5378=AXIS2_PLACEMENT_3D ( 'NONE', #93095, #3409, #80040 ) ;
#5379=CARTESIAN_POINT ( 'NONE',  ( -12.29999999999999538, 2.500000000000000000, 4.576537180435972019 ) ) ;
#5380=CARTESIAN_POINT ( 'NONE',  ( -6.700000000000019718, 2.500000000000000000, -4.330127018922201643 ) ) ;
#5381=EDGE_CURVE ( 'NONE', #108643, #69133, #27668, .T. ) ;
#5382=CARTESIAN_POINT ( 'NONE',  ( 6.049999999999934097, 2.500000000000000000, -6.048780366869526581 ) ) ;
#5383=ORIENTED_EDGE ( 'NONE', *, *, #102734, .F. ) ;
#5384=EDGE_CURVE ( 'NONE', #74183, #78070, #42608, .T. ) ;
#5385=CARTESIAN_POINT ( 'NONE',  ( -2.050000000000032685, 12.50000000000000000, -2.165063509461101710 ) ) ;
#5386=EDGE_CURVE ( 'NONE', #109254, #126002, #36351, .T. ) ;
#5387=ORIENTED_EDGE ( 'NONE', *, *, #73660, .T. ) ;
#5388=FACE_OUTER_BOUND ( 'NONE', #75262, .T. ) ;
#5389=EDGE_CURVE ( 'NONE', #60649, #91248, #57258, .T. ) ;
#5390=ORIENTED_EDGE ( 'NONE', *, *, #26232, .F. ) ;
#5391=CARTESIAN_POINT ( 'NONE',  ( -5.850000000000021849, 12.50000000000000000, -2.857883832488653741 ) ) ;
#5392=ORIENTED_EDGE ( 'NONE', *, *, #73708, .T. ) ;
#5393=ORIENTED_EDGE ( 'NONE', *, *, #15700, .F. ) ;
#5394=EDGE_CURVE ( 'NONE', #31364, #12823, #61375, .T. ) ;
#5395=DIRECTION ( 'NONE',  ( 0.000000000000000000, 1.000000000000000000, 0.000000000000000000 ) ) ;
#5396=CARTESIAN_POINT ( 'NONE',  ( 17.50000000000000000, -2.500000000000000000, 0.000000000000000000 ) ) ;
#5397=AXIS2_PLACEMENT_3D ( 'NONE', #92593, #54579, #4187 ) ;
#5398=CIRCLE ( 'NONE', #59719, 0.06509327318403745899 ) ;
#5399=CARTESIAN_POINT ( 'NONE',  ( -11.64999999999999858, 2.500000000000000000, -1.472243186433546125 ) ) ;
#5400=CARTESIAN_POINT ( 'NONE',  ( -7.500000000000016875, 2.500000000000000000, 0.6928203230275494784 ) ) ;
#5401=ORIENTED_EDGE ( 'NONE', *, *, #47169, .T. ) ;
#5402=CARTESIAN_POINT ( 'NONE',  ( 7.499999999999961808, 2.500000000000000000, -4.430127018922202176 ) ) ;
#5403=CARTESIAN_POINT ( 'NONE',  ( -10.40000000000000213, 12.50000000000000000, 3.637306695894644726 ) ) ;
#5404=CARTESIAN_POINT ( 'NONE',  ( -5.650000000000023448, 2.500000000000000000, -6.148780366869526226 ) ) ;
#5406=DIRECTION ( 'NONE',  ( 0.000000000000000000, 0.000000000000000000, 1.000000000000000000 ) ) ;
#5407=ORIENTED_EDGE ( 'NONE', *, *, #100584, .F. ) ;
#5408=ORIENTED_EDGE ( 'NONE', *, *, #23703, .F. ) ;
#5409=AXIS2_PLACEMENT_3D ( 'NONE', #91243, #89943, #40214 ) ;
#5410=ORIENTED_EDGE ( 'NONE', *, *, #22969, .F. ) ;
#5411=VECTOR ( 'NONE', #46133, 1000.000000000000000 ) ;
#5412=CARTESIAN_POINT ( 'NONE',  ( 0.7999999999999548583, 12.50000000000000000, 4.330127018922196314 ) ) ;
#5413=DIRECTION ( 'NONE',  ( 0.000000000000000000, 1.000000000000000000, 0.000000000000000000 ) ) ;
#5414=AXIS2_PLACEMENT_3D ( 'NONE', #127686, #60266, #88390 ) ;
#5415=AXIS2_PLACEMENT_3D ( 'NONE', #54207, #124236, #43758 ) ;
#5417=CARTESIAN_POINT ( 'NONE',  ( 7.499999999999925393, 12.50000000000000000, -0.6277270498435166823 ) ) ;
#5418=DIRECTION ( 'NONE',  ( 0.000000000000000000, 1.000000000000000000, 0.000000000000000000 ) ) ;
#5419=CARTESIAN_POINT ( 'NONE',  ( 13.29999999999990301, 12.50000000000000000, -4.395220292106239768 ) ) ;
#5420=CARTESIAN_POINT ( 'NONE',  ( 9.399999999999915090, 12.50000000000000000, -4.048810130592463530 ) ) ;
#5421=ORIENTED_EDGE ( 'NONE', *, *, #48546, .F. ) ;
#5422=ADVANCED_FACE ( 'NONE', ( #78080 ), #30088, .T. ) ;
#5423=DIRECTION ( 'NONE',  ( -0.000000000000000000, 1.000000000000000000, -0.000000000000000000 ) ) ;
#5424=DIRECTION ( 'NONE',  ( 0.000000000000000000, 0.000000000000000000, 1.000000000000000000 ) ) ;
#5425=EDGE_CURVE ( 'NONE', #106738, #8949, #13324, .T. ) ;
#5426=ORIENTED_EDGE ( 'NONE', *, *, #104379, .F. ) ;
#5427=CARTESIAN_POINT ( 'NONE',  ( 3.949999999999938893, 2.500000000000000000, 6.248780366869520542 ) ) ;
#5428=CIRCLE ( 'NONE', #107846, 0.06509327318403745899 ) ;
#5429=DIRECTION ( 'NONE',  ( -0.000000000000000000, 1.000000000000000000, -0.000000000000000000 ) ) ;
#5430=DIRECTION ( 'NONE',  ( 0.000000000000000000, 1.000000000000000000, 0.000000000000000000 ) ) ;
#5431=ORIENTED_EDGE ( 'NONE', *, *, #128653, .F. ) ;
#5432=DIRECTION ( 'NONE',  ( -0.000000000000000000, -1.000000000000000000, -0.000000000000000000 ) ) ;
#5434=ORIENTED_EDGE ( 'NONE', *, *, #114585, .F. ) ;
#5435=DIRECTION ( 'NONE',  ( 0.000000000000000000, 1.000000000000000000, 0.000000000000000000 ) ) ;
#5436=CARTESIAN_POINT ( 'NONE',  ( 2.299999999999948752, 12.50000000000000000, -4.048810130592463530 ) ) ;
#5437=FACE_OUTER_BOUND ( 'NONE', #80381, .T. ) ;
#5438=CONICAL_SURFACE ( 'NONE', #89085, 0.1000000000000000056, 0.003490658503988666988 ) ;
#5439=AXIS2_PLACEMENT_3D ( 'NONE', #46696, #66324, #95792 ) ;
#5440=EDGE_LOOP ( 'NONE', ( #82980, #17495, #65727, #30628 ) ) ;
#5441=VECTOR ( 'NONE', #109964, 1000.000000000000000 ) ;
#5442=DIRECTION ( 'NONE',  ( 0.000000000000000000, 0.000000000000000000, -1.000000000000000000 ) ) ;
#5443=EDGE_LOOP ( 'NONE', ( #25934, #36081, #118557, #2574 ) ) ;
#5444=CARTESIAN_POINT ( 'NONE',  ( -12.49999999999999289, 2.500000000000000000, -4.922947341949750921 ) ) ;
#5445=AXIS2_PLACEMENT_3D ( 'NONE', #446, #77722, #87550 ) ;
#5446=EDGE_LOOP ( 'NONE', ( #33661, #95263 ) ) ;
#5447=AXIS2_PLACEMENT_3D ( 'NONE', #83761, #114500, #82490 ) ;
#5449=ORIENTED_EDGE ( 'NONE', *, *, #83683, .F. ) ;
#5450=CARTESIAN_POINT ( 'NONE',  ( -11.44999999999999751, 12.50000000000000000, -6.841600689897074261 ) ) ;
#5451=LINE ( 'NONE', #44756, #81385 ) ;
#5452=VERTEX_POINT ( 'NONE', #47986 ) ;
#5453=DIRECTION ( 'NONE',  ( -0.000000000000000000, -1.000000000000000000, -0.000000000000000000 ) ) ;
#5454=CARTESIAN_POINT ( 'NONE',  ( -7.100000000000017408, 12.50000000000000000, 0.6928203230275494784 ) ) ;
#5455=EDGE_LOOP ( 'NONE', ( #4785, #9220 ) ) ;
#5456=DIRECTION ( 'NONE',  ( 0.000000000000000000, 0.000000000000000000, 1.000000000000000000 ) ) ;
#5457=EDGE_CURVE ( 'NONE', #11223, #14873, #813, .T. ) ;
#5458=DIRECTION ( 'NONE',  ( -0.000000000000000000, 1.000000000000000000, -0.000000000000000000 ) ) ;
#5459=FACE_OUTER_BOUND ( 'NONE', #232, .T. ) ;
#5460=DIRECTION ( 'NONE',  ( 0.000000000000000000, 0.000000000000000000, -1.000000000000000000 ) ) ;
#5461=DIRECTION ( 'NONE',  ( 0.000000000000000000, -0.9999939076577903929, 0.003490651415223739937 ) ) ;
#5462=DIRECTION ( 'NONE',  ( -0.000000000000000000, -1.000000000000000000, -0.000000000000000000 ) ) ;
#5463=ORIENTED_EDGE ( 'NONE', *, *, #4933, .F. ) ;
#5464=VERTEX_POINT ( 'NONE', #126541 ) ;
#5465=ORIENTED_EDGE ( 'NONE', *, *, #43572, .T. ) ;
#5466=ORIENTED_EDGE ( 'NONE', *, *, #19965, .F. ) ;
#5467=CARTESIAN_POINT ( 'NONE',  ( 43.29488422903774847, 3.510951914389877526, 3.940494739282152992 ) ) ;
#5468=DIRECTION ( 'NONE',  ( 0.000000000000000000, 0.000000000000000000, 1.000000000000000000 ) ) ;
#5469=EDGE_CURVE ( 'NONE', #51819, #118832, #84447, .T. ) ;
#5470=DIRECTION ( 'NONE',  ( -0.000000000000000000, -1.000000000000000000, -0.000000000000000000 ) ) ;
#5471=ORIENTED_EDGE ( 'NONE', *, *, #73353, .F. ) ;
#5472=FACE_BOUND ( 'NONE', #62179, .T. ) ;
#5473=ADVANCED_FACE ( 'NONE', ( #117991 ), #108335, .T. ) ;
#5474=DIRECTION ( 'NONE',  ( -0.000000000000000000, -1.000000000000000000, -0.000000000000000000 ) ) ;
#5475=CARTESIAN_POINT ( 'NONE',  ( 4.999999999999936939, 12.50000000000000000, -3.637306695894650055 ) ) ;
#5476=CARTESIAN_POINT ( 'NONE',  ( -1.650000000000034772, 2.500000000000000000, 2.065063509461097624 ) ) ;
#5477=CIRCLE ( 'NONE', #91179, 0.1000000000000002554 ) ;
#5478=CARTESIAN_POINT ( 'NONE',  ( -8.350000000000012079, 2.500000000000000000, -2.857883832488653741 ) ) ;
#5479=CARTESIAN_POINT ( 'NONE',  ( -3.642919299551294898E-14, 2.500000000000000000, 0.6928203230275518099 ) ) ;
#5480=DIRECTION ( 'NONE',  ( -0.000000000000000000, -1.000000000000000000, -0.000000000000000000 ) ) ;
#5481=CARTESIAN_POINT ( 'NONE',  ( 0.000000000000000000, 12.50000000000000000, 0.06509327318403743123 ) ) ;
#5482=DIRECTION ( 'NONE',  ( 0.000000000000000000, 0.000000000000000000, 1.000000000000000000 ) ) ;
#5483=EDGE_CURVE ( 'NONE', #11815, #117684, #47339, .T. ) ;
#5484=CARTESIAN_POINT ( 'NONE',  ( -0.6000000000000383915, 2.500000000000000000, -3.883716857408426648 ) ) ;
#5485=DIRECTION ( 'NONE',  ( 0.000000000000000000, -0.9999939076577903929, 0.003490651415223739937 ) ) ;
#5486=VECTOR ( 'NONE', #124407, 1000.000000000000000 ) ;
#5487=CIRCLE ( 'NONE', #72413, 0.09999999999999982514 ) ;
#5488=ORIENTED_EDGE ( 'NONE', *, *, #115000, .F. ) ;
#5489=VERTEX_POINT ( 'NONE', #28341 ) ;
#5490=VERTEX_POINT ( 'NONE', #8033 ) ;
#5491=ORIENTED_EDGE ( 'NONE', *, *, #24041, .F. ) ;
#5492=CARTESIAN_POINT ( 'NONE',  ( 7.899999999999924860, 2.500000000000000000, 5.022947341949748790 ) ) ;
#5493=ORIENTED_EDGE ( 'NONE', *, *, #83409, .F. ) ;
#5494=DIRECTION ( 'NONE',  ( -0.000000000000000000, 1.000000000000000000, -0.000000000000000000 ) ) ;
#5495=ORIENTED_EDGE ( 'NONE', *, *, #9273, .F. ) ;
#5496=VERTEX_POINT ( 'NONE', #58452 ) ;
#5497=CARTESIAN_POINT ( 'NONE',  ( 9.549999999999915445, 2.500000000000000000, 6.595190528383296780 ) ) ;
#5498=CIRCLE ( 'NONE', #55683, 0.1000000000000000472 ) ;
#5499=AXIS2_PLACEMENT_3D ( 'NONE', #64216, #56321, #123766 ) ;
#5500=CARTESIAN_POINT ( 'NONE',  ( 8.920123399940051101, -2.500000000000000444, 8.410822907403851190 ) ) ;
#5501=CARTESIAN_POINT ( 'NONE',  ( 6.249999999999932498, 12.50000000000000000, -2.922977105672691422 ) ) ;
#5502=DIRECTION ( 'NONE',  ( 0.000000000000000000, 1.000000000000000000, 0.000000000000000000 ) ) ;
#5503=CARTESIAN_POINT ( 'NONE',  ( -4.400000000000025224, 12.50000000000000000, 0.2813168883297361700 ) ) ;
#5504=VERTEX_POINT ( 'NONE', #89186 ) ;
#5505=ORIENTED_EDGE ( 'NONE', *, *, #127912, .T. ) ;
#5506=ADVANCED_FACE ( 'NONE', ( #39470 ), #79377, .T. ) ;
#5507=ORIENTED_EDGE ( 'NONE', *, *, #118386, .F. ) ;
#5508=CARTESIAN_POINT ( 'NONE',  ( 14.14999999999989377, 2.500000000000000000, -1.572243186433550211 ) ) ;
#5509=ORIENTED_EDGE ( 'NONE', *, *, #6716, .F. ) ;
#5510=CARTESIAN_POINT ( 'NONE',  ( -10.00000000000000711, 12.50000000000000000, -3.637306695894645614 ) ) ;
#5511=ORIENTED_EDGE ( 'NONE', *, *, #12211, .T. ) ;
#5512=ADVANCED_FACE ( 'NONE', ( #70193 ), #71465, .T. ) ;
#5513=VECTOR ( 'NONE', #87593, 1000.000000000000000 ) ;
#5514=ORIENTED_EDGE ( 'NONE', *, *, #64965, .F. ) ;
#5515=EDGE_CURVE ( 'NONE', #74476, #93079, #41558, .T. ) ;
#5516=PLANE ( 'NONE',  #67287 ) ;
#5517=DIRECTION ( 'NONE',  ( 0.000000000000000000, 0.000000000000000000, 1.000000000000000000 ) ) ;
#5518=LINE ( 'NONE', #26475, #95968 ) ;
#5519=CIRCLE ( 'NONE', #64029, 0.06509327318403745899 ) ;
#5520=FACE_OUTER_BOUND ( 'NONE', #107670, .T. ) ;
#5521=EDGE_CURVE ( 'NONE', #74712, #2890, #70780, .T. ) ;
#5522=ADVANCED_FACE ( 'NONE', ( #121220 ), #120951, .T. ) ;
#5523=DIRECTION ( 'NONE',  ( 0.000000000000000000, -0.9999939076577903929, 0.003490651415223739937 ) ) ;
#5524=AXIS2_PLACEMENT_3D ( 'NONE', #65380, #105321, #63467 ) ;
#5525=DIRECTION ( 'NONE',  ( 0.000000000000000000, 1.000000000000000000, 0.000000000000000000 ) ) ;
#5526=EDGE_CURVE ( 'NONE', #93332, #51670, #51211, .T. ) ;
#5527=CONICAL_SURFACE ( 'NONE', #49482, 0.1000000000000002554, 0.003490658503988666988 ) ;
#5528=EDGE_CURVE ( 'NONE', #53090, #88981, #16370, .T. ) ;
#5529=ORIENTED_EDGE ( 'NONE', *, *, #88308, .F. ) ;
#5530=DIRECTION ( 'NONE',  ( -0.000000000000000000, -1.000000000000000000, -0.000000000000000000 ) ) ;
#5532=EDGE_LOOP ( 'NONE', ( #127885, #101640, #123823, #118707 ) ) ;
#5533=CONICAL_SURFACE ( 'NONE', #80781, 0.1000000000000000472, 0.003490658503988666988 ) ;
#5534=CARTESIAN_POINT ( 'NONE',  ( -0.4000000000000404898, 12.50000000000000000, 5.022947341949748790 ) ) ;
#5535=EDGE_CURVE ( 'NONE', #123894, #69676, #2725, .T. ) ;
#5536=VERTEX_POINT ( 'NONE', #121863 ) ;
#5537=DIRECTION ( 'NONE',  ( 0.000000000000000000, 1.000000000000000000, 0.000000000000000000 ) ) ;
#5538=DIRECTION ( 'NONE',  ( 0.000000000000000000, 0.000000000000000000, 1.000000000000000000 ) ) ;
#5539=EDGE_LOOP ( 'NONE', ( #103673, #78625 ) ) ;
#5540=DIRECTION ( 'NONE',  ( 0.000000000000000000, 0.000000000000000000, 1.000000000000000000 ) ) ;
#5541=CARTESIAN_POINT ( 'NONE',  ( -7.499999999999980460, 2.500000000000000000, -4.330127018922201643 ) ) ;
#5542=ORIENTED_EDGE ( 'NONE', *, *, #119028, .F. ) ;
#5543=EDGE_CURVE ( 'NONE', #56755, #102028, #83321, .T. ) ;
#5544=AXIS2_PLACEMENT_3D ( 'NONE', #28657, #68557, #108483 ) ;
#5545=CARTESIAN_POINT ( 'NONE',  ( -5.850000000000022737, 2.500000000000000000, -6.495190528383302464 ) ) ;
#5546=AXIS2_PLACEMENT_3D ( 'NONE', #100033, #41129, #49012 ) ;
#5547=VECTOR ( 'NONE', #26280, 1000.000000000000000 ) ;
#5548=CARTESIAN_POINT ( 'NONE',  ( -13.14999999999999147, 2.500000000000000000, -2.511473670974875727 ) ) ;
#5549=EDGE_LOOP ( 'NONE', ( #109464, #5364 ) ) ;
#5550=VERTEX_POINT ( 'NONE', #60393 ) ;
#5551=ORIENTED_EDGE ( 'NONE', *, *, #18503, .F. ) ;
#5552=DIRECTION ( 'NONE',  ( 0.000000000000000000, -0.000000000000000000, 1.000000000000000000 ) ) ;
#5553=CARTESIAN_POINT ( 'NONE',  ( 0.4499999999999569344, 2.500000000000000000, -2.165063509461101710 ) ) ;
#5555=CARTESIAN_POINT ( 'NONE',  ( -3.100000000000028955, 2.500000000000000000, 3.883716857408421319 ) ) ;
#5556=FACE_OUTER_BOUND ( 'NONE', #114193, .T. ) ;
#5557=CARTESIAN_POINT ( 'NONE',  ( 12.09999999999990550, 12.50000000000000000, -3.637306695894650055 ) ) ;
#5559=CARTESIAN_POINT ( 'NONE',  ( 14.99999999999989342, 12.50000000000000000, -0.6928203230275541413 ) ) ;
#5560=EDGE_LOOP ( 'NONE', ( #90102, #83229 ) ) ;
#5561=DIRECTION ( 'NONE',  ( 0.000000000000000000, 0.000000000000000000, -1.000000000000000000 ) ) ;
#5562=LINE ( 'NONE', #46147, #4688 ) ;
#5563=DIRECTION ( 'NONE',  ( 0.000000000000000000, 1.000000000000000000, 0.000000000000000000 ) ) ;
#5564=ORIENTED_EDGE ( 'NONE', *, *, #90344, .F. ) ;
#5565=EDGE_CURVE ( 'NONE', #126422, #97481, #24812, .T. ) ;
#5566=VECTOR ( 'NONE', #66745, 1000.000000000000000 ) ;
#5567=DIRECTION ( 'NONE',  ( 0.000000000000000000, 0.000000000000000000, 1.000000000000000000 ) ) ;
#5568=CARTESIAN_POINT ( 'NONE',  ( -12.69999999999999218, 2.500000000000000000, -0.3464101615137741286 ) ) ;
#5569=ORIENTED_EDGE ( 'NONE', *, *, #56895, .T. ) ;
#5570=AXIS2_PLACEMENT_3D ( 'NONE', #66478, #85484, #109477 ) ;
#5571=DIRECTION ( 'NONE',  ( -0.000000000000000000, -1.000000000000000000, -0.000000000000000000 ) ) ;
#5572=ADVANCED_FACE ( 'NONE', ( #90455 ), #58271, .T. ) ;
#5573=ORIENTED_EDGE ( 'NONE', *, *, #25416, .F. ) ;
#5574=ORIENTED_EDGE ( 'NONE', *, *, #47275, .T. ) ;
#5575=DIRECTION ( 'NONE',  ( 0.000000000000000000, 0.000000000000000000, -1.000000000000000000 ) ) ;
#5576=VECTOR ( 'NONE', #104191, 1000.000000000000000 ) ;
#5577=EDGE_LOOP ( 'NONE', ( #53434, #67594, #88455, #29839 ) ) ;
#5578=DIRECTION ( 'NONE',  ( 0.000000000000000000, 0.000000000000000000, -1.000000000000000000 ) ) ;
#5579=CARTESIAN_POINT ( 'NONE',  ( -7.499999999999976907, 2.500000000000000000, 4.230127018922196669 ) ) ;
#5580=CIRCLE ( 'NONE', #72519, 0.1000000000000000472 ) ;
#5581=AXIS2_PLACEMENT_3D ( 'NONE', #17009, #127024, #119125 ) ;
#5582=CARTESIAN_POINT ( 'NONE',  ( -12.49999999999995737, 2.500000000000000000, 4.330127018922196314 ) ) ;
#5583=EDGE_LOOP ( 'NONE', ( #28892, #44647, #32509, #111013 ) ) ;
#5584=CONICAL_SURFACE ( 'NONE', #85016, 0.1000000000000002554, 0.003490658503988666988 ) ;
#5585=FACE_BOUND ( 'NONE', #41124, .T. ) ;
#5586=DIRECTION ( 'NONE',  ( 0.000000000000000000, -0.9999939076577903929, 0.003490651415223739937 ) ) ;
#5587=ORIENTED_EDGE ( 'NONE', *, *, #27303, .F. ) ;
#5588=DIRECTION ( 'NONE',  ( 0.000000000000000000, 0.000000000000000000, 1.000000000000000000 ) ) ;
#5589=CARTESIAN_POINT ( 'NONE',  ( -12.29999999999999538, 2.500000000000000000, -4.676537180435976104 ) ) ;
#5590=EDGE_LOOP ( 'NONE', ( #74348, #85355 ) ) ;
#5591=ORIENTED_EDGE ( 'NONE', *, *, #38964, .T. ) ;
#5592=EDGE_LOOP ( 'NONE', ( #31315, #68551, #67878, #8634 ) ) ;
#5593=DIRECTION ( 'NONE',  ( 0.000000000000000000, -0.000000000000000000, 1.000000000000000000 ) ) ;
#5594=DIRECTION ( 'NONE',  ( 0.000000000000000000, 0.000000000000000000, -1.000000000000000000 ) ) ;
#5595=DIRECTION ( 'NONE',  ( -0.000000000000000000, -1.000000000000000000, -0.000000000000000000 ) ) ;
#5596=FACE_BOUND ( 'NONE', #58620, .T. ) ;
#5597=EDGE_LOOP ( 'NONE', ( #10928, #123348 ) ) ;
#5598=AXIS2_PLACEMENT_3D ( 'NONE', #25964, #75058, #63951 ) ;
#5600=AXIS2_PLACEMENT_3D ( 'NONE', #66825, #65552, #36758 ) ;
#5601=CARTESIAN_POINT ( 'NONE',  ( -7.050000000000016698, 2.500000000000000000, -2.065063509461102065 ) ) ;
#5602=CARTESIAN_POINT ( 'NONE',  ( 2.099999999999948574, 2.500000000000000000, 4.430127018922196847 ) ) ;
#5603=AXIS2_PLACEMENT_3D ( 'NONE', #100966, #11296, #51252 ) ;
#5604=ADVANCED_FACE ( 'NONE', ( #51849 ), #49928, .T. ) ;
#5605=DIRECTION ( 'NONE',  ( -0.000000000000000000, -1.000000000000000000, -0.000000000000000000 ) ) ;
#5606=AXIS2_PLACEMENT_3D ( 'NONE', #104923, #15247, #5442 ) ;
#5607=LINE ( 'NONE', #46856, #61114 ) ;
#5609=CARTESIAN_POINT ( 'NONE',  ( 0.8499999999999553468, 12.50000000000000000, -2.922977105672691422 ) ) ;
#5610=VECTOR ( 'NONE', #117501, 1000.000000000000000 ) ;
#5611=CARTESIAN_POINT ( 'NONE',  ( 16.55874544816223448, 0.4845305829267578801, 6.091953208799004926 ) ) ;
#5612=CONICAL_SURFACE ( 'NONE', #110096, 0.1000000000000002554, 0.003490658503988666988 ) ;
#5613=EDGE_CURVE ( 'NONE', #49210, #10571, #87490, .T. ) ;
#5614=FACE_OUTER_BOUND ( 'NONE', #128737, .T. ) ;
#5615=AXIS2_PLACEMENT_3D ( 'NONE', #21704, #1400, #109432 ) ;
#5617=ORIENTED_EDGE ( 'NONE', *, *, #118129, .T. ) ;
#5618=VERTEX_POINT ( 'NONE', #9980 ) ;
#5619=EDGE_LOOP ( 'NONE', ( #118635, #70062, #16081, #106205 ) ) ;
#5620=EDGE_LOOP ( 'NONE', ( #50477, #23687 ) ) ;
#5621=DIRECTION ( 'NONE',  ( 0.000000000000000000, 0.000000000000000000, 1.000000000000000000 ) ) ;
#5622=EDGE_CURVE ( 'NONE', #94894, #40952, #2078, .T. ) ;
#5623=PLANE ( 'NONE',  #4816 ) ;
#5624=AXIS2_PLACEMENT_3D ( 'NONE', #127701, #8554, #77955 ) ;
#5625=ORIENTED_EDGE ( 'NONE', *, *, #89977, .T. ) ;
#5626=FACE_BOUND ( 'NONE', #115042, .T. ) ;
#5627=ADVANCED_FACE ( 'NONE', ( #42022 ), #100035, .T. ) ;
#5628=CIRCLE ( 'NONE', #55822, 0.06509327318403745899 ) ;
#5629=LINE ( 'NONE', #122845, #8057 ) ;
#5630=AXIS2_PLACEMENT_3D ( 'NONE', #65238, #105173, #85538 ) ;
#5631=AXIS2_PLACEMENT_3D ( 'NONE', #113858, #96770, #86964 ) ;
#5632=EDGE_CURVE ( 'NONE', #41715, #21708, #40756, .T. ) ;
#5633=CARTESIAN_POINT ( 'NONE',  ( -7.700000000000016165, 12.50000000000000000, -3.983716857408426293 ) ) ;
#5634=EDGE_LOOP ( 'NONE', ( #12952, #108098, #38152, #117411 ) ) ;
#5635=PLANE ( 'NONE',  #128998 ) ;
#5636=CARTESIAN_POINT ( 'NONE',  ( 11.64999999999990443, 12.50000000000000000, 2.857883832488649301 ) ) ;
#5638=LINE ( 'NONE', #64566, #32947 ) ;
#5639=EDGE_LOOP ( 'NONE', ( #69738, #28016 ) ) ;
#5640=CARTESIAN_POINT ( 'NONE',  ( 0.6499999999999561684, 2.500000000000000000, 2.611473670974873151 ) ) ;
#5641=ORIENTED_EDGE ( 'NONE', *, *, #122178, .T. ) ;
#5642=ORIENTED_EDGE ( 'NONE', *, *, #19648, .T. ) ;
#5643=ORIENTED_EDGE ( 'NONE', *, *, #102488, .F. ) ;
#5644=FACE_OUTER_BOUND ( 'NONE', #22816, .T. ) ;
#5645=DIRECTION ( 'NONE',  ( 0.000000000000000000, -0.9999939076577903929, 0.003490651415223739937 ) ) ;
#5646=CARTESIAN_POINT ( 'NONE',  ( -7.500000000000016875, 2.500000000000000000, -3.637306695894650055 ) ) ;
#5647=ORIENTED_EDGE ( 'NONE', *, *, #47338, .F. ) ;
#5648=CIRCLE ( 'NONE', #110126, 0.06509327318403745899 ) ;
#5649=CARTESIAN_POINT ( 'NONE',  ( 14.93814515115542640, 2.500000000000000444, -6.173787963789177269 ) ) ;
#5650=FACE_OUTER_BOUND ( 'NONE', #97587, .T. ) ;
#5651=CARTESIAN_POINT ( 'NONE',  ( -1.050000000000037792, 2.500000000000000000, 1.718653347947321386 ) ) ;
#5653=CARTESIAN_POINT ( 'NONE',  ( -15.59999999999998010, 12.50000000000000000, -0.2813168883297385570 ) ) ;
#5654=DIRECTION ( 'NONE',  ( -4.274815082592931898E-19, -0.9999939076577903929, -0.003490651415223739937 ) ) ;
#5655=ORIENTED_EDGE ( 'NONE', *, *, #26530, .F. ) ;
#5656=DIRECTION ( 'NONE',  ( -0.000000000000000000, 1.000000000000000000, -0.000000000000000000 ) ) ;
#5657=CONICAL_SURFACE ( 'NONE', #87144, 0.09999999999999982514, 0.003490658503988666988 ) ;
#5658=ORIENTED_EDGE ( 'NONE', *, *, #84490, .T. ) ;
#5659=VECTOR ( 'NONE', #97824, 1000.000000000000000 ) ;
#5660=ORIENTED_EDGE ( 'NONE', *, *, #38584, .F. ) ;
#5661=FACE_OUTER_BOUND ( 'NONE', #127077, .T. ) ;
#5662=CARTESIAN_POINT ( 'NONE',  ( -10.80000000000000071, 12.50000000000000000, -0.06509327318403970719 ) ) ;
#5663=DIRECTION ( 'NONE',  ( -0.000000000000000000, 1.000000000000000000, -0.000000000000000000 ) ) ;
#5664=DIRECTION ( 'NONE',  ( -0.000000000000000000, -1.000000000000000000, -0.000000000000000000 ) ) ;
#5665=EDGE_LOOP ( 'NONE', ( #1876, #2474, #35663, #9585 ) ) ;
#5666=AXIS2_PLACEMENT_3D ( 'NONE', #76590, #66117, #96211 ) ;
#5668=ORIENTED_EDGE ( 'NONE', *, *, #87969, .F. ) ;
#5669=EDGE_CURVE ( 'NONE', #83259, #61624, #43609, .T. ) ;
#5670=FACE_OUTER_BOUND ( 'NONE', #95957, .T. ) ;
#5671=LINE ( 'NONE', #45633, #64136 ) ;
#5672=CARTESIAN_POINT ( 'NONE',  ( -5.400000000000023448, 12.50000000000000000, -4.265033745738164406 ) ) ;
#5673=EDGE_CURVE ( 'NONE', #124518, #87255, #18459, .T. ) ;
#5674=EDGE_LOOP ( 'NONE', ( #34941, #64826, #29441, #115671 ) ) ;
#5675=EDGE_LOOP ( 'NONE', ( #114849, #35240, #55808, #8326 ) ) ;
#5676=EDGE_CURVE ( 'NONE', #119267, #40041, #12177, .T. ) ;
#5677=DIRECTION ( 'NONE',  ( 0.000000000000000000, 0.000000000000000000, 1.000000000000000000 ) ) ;
#5678=ADVANCED_FACE ( 'NONE', ( #70044 ), #74904, .T. ) ;
#5679=AXIS2_PLACEMENT_3D ( 'NONE', #41665, #81564, #72401 ) ;
#5680=VECTOR ( 'NONE', #63427, 1000.000000000000000 ) ;
#5681=EDGE_CURVE ( 'NONE', #40822, #9001, #85359, .T. ) ;
#5683=CARTESIAN_POINT ( 'NONE',  ( -1.450000000000035483, 2.500000000000000000, 6.048780366869521252 ) ) ;
#5684=AXIS2_PLACEMENT_3D ( 'NONE', #31576, #72791, #115248 ) ;
#5685=DIRECTION ( 'NONE',  ( -0.000000000000000000, -1.000000000000000000, -0.000000000000000000 ) ) ;
#5686=ORIENTED_EDGE ( 'NONE', *, *, #82605, .F. ) ;
#5687=DIRECTION ( 'NONE',  ( 0.000000000000000000, -0.9999939076577903929, 0.003490651415223739937 ) ) ;
#5688=EDGE_CURVE ( 'NONE', #18148, #59490, #22243, .T. ) ;
#5689=DIRECTION ( 'NONE',  ( 0.000000000000000000, 1.000000000000000000, 0.000000000000000000 ) ) ;
#5690=CARTESIAN_POINT ( 'NONE',  ( 9.999999999999912959, 12.50000000000000000, -5.022947341949754119 ) ) ;
#5691=DIRECTION ( 'NONE',  ( 0.000000000000000000, 1.000000000000000000, 0.000000000000000000 ) ) ;
#5692=ORIENTED_EDGE ( 'NONE', *, *, #7555, .T. ) ;
#5693=EDGE_CURVE ( 'NONE', #73131, #69690, #79116, .T. ) ;
#5694=CARTESIAN_POINT ( 'NONE',  ( -1.050000000000038680, 2.500000000000000000, 6.941600689897073018 ) ) ;
#5695=ADVANCED_FACE ( 'NONE', ( #640 ), #45665, .T. ) ;
#5696=CARTESIAN_POINT ( 'NONE',  ( -13.54999999999998828, 12.50000000000000000, 1.753560074763288013 ) ) ;
#5697=VERTEX_POINT ( 'NONE', #80518 ) ;
#5698=ORIENTED_EDGE ( 'NONE', *, *, #34163, .T. ) ;
#5701=DIRECTION ( 'NONE',  ( 0.000000000000000000, 0.000000000000000000, 1.000000000000000000 ) ) ;
#5702=DIRECTION ( 'NONE',  ( -0.000000000000000000, 1.000000000000000000, -0.000000000000000000 ) ) ;
#5703=AXIS2_PLACEMENT_3D ( 'NONE', #123040, #13706, #92940 ) ;
#5704=DIRECTION ( 'NONE',  ( -4.274815082592931898E-19, -0.9999939076577903929, -0.003490651415223739937 ) ) ;
#5705=AXIS2_PLACEMENT_3D ( 'NONE', #78392, #48930, #99952 ) ;
#5706=CARTESIAN_POINT ( 'NONE',  ( -5.850000000000019185, 2.500000000000000000, 6.395190528383296602 ) ) ;
#5708=DIRECTION ( 'NONE',  ( -0.000000000000000000, 1.000000000000000000, -0.000000000000000000 ) ) ;
#5709=DIRECTION ( 'NONE',  ( 0.000000000000000000, 1.000000000000000000, 0.000000000000000000 ) ) ;
#5710=CARTESIAN_POINT ( 'NONE',  ( -5.200000000000022382, 2.500000000000000000, 0.3464101615137735735 ) ) ;
#5711=VECTOR ( 'NONE', #51551, 1000.000000000000000 ) ;
#5712=CARTESIAN_POINT ( 'NONE',  ( 7.949999999999925571, 2.500000000000000000, 2.165063509461097713 ) ) ;
#5713=VERTEX_POINT ( 'NONE', #64083 ) ;
#5714=CIRCLE ( 'NONE', #3383, 0.09999999999999982514 ) ;
#5715=EDGE_LOOP ( 'NONE', ( #89701, #33061 ) ) ;
#5716=EDGE_LOOP ( 'NONE', ( #89197, #62835 ) ) ;
#5717=CIRCLE ( 'NONE', #60046, 0.1000000000000002554 ) ;
#5718=DIRECTION ( 'NONE',  ( 0.000000000000000000, 0.000000000000000000, 1.000000000000000000 ) ) ;
#5719=DIRECTION ( 'NONE',  ( 0.000000000000000000, 1.000000000000000000, 0.000000000000000000 ) ) ;
#5720=VERTEX_POINT ( 'NONE', #54266 ) ;
#5721=DIRECTION ( 'NONE',  ( 0.000000000000000000, -0.9999939076577903929, 0.003490651415223739937 ) ) ;
#5722=AXIS2_PLACEMENT_3D ( 'NONE', #86668, #104383, #84084 ) ;
#5723=VECTOR ( 'NONE', #124148, 1000.000000000000000 ) ;
#5724=DIRECTION ( 'NONE',  ( 0.000000000000000000, 0.000000000000000000, 1.000000000000000000 ) ) ;
#5725=DIRECTION ( 'NONE',  ( 0.000000000000000000, 1.000000000000000000, 0.000000000000000000 ) ) ;
#5726=ORIENTED_EDGE ( 'NONE', *, *, #65688, .T. ) ;
#5727=DIRECTION ( 'NONE',  ( 0.000000000000000000, -0.000000000000000000, 1.000000000000000000 ) ) ;
#5728=EDGE_LOOP ( 'NONE', ( #91786, #44566, #127705, #72618 ) ) ;
#5729=ADVANCED_FACE ( 'NONE', ( #103370 ), #28939, .T. ) ;
#5730=EDGE_LOOP ( 'NONE', ( #99024, #116232, #75971, #65661 ) ) ;
#5731=ORIENTED_EDGE ( 'NONE', *, *, #34651, .T. ) ;
#5732=ORIENTED_EDGE ( 'NONE', *, *, #114540, .T. ) ;
#5733=CARTESIAN_POINT ( 'NONE',  ( -0.4000000000000392131, 2.500000000000000000, -4.330127018922201643 ) ) ;
#5734=CARTESIAN_POINT ( 'NONE',  ( 9.349999999999919709, 2.500000000000000000, 2.511473670974873507 ) ) ;
#5735=DIRECTION ( 'NONE',  ( 0.000000000000000000, 0.000000000000000000, 1.000000000000000000 ) ) ;
#5736=CARTESIAN_POINT ( 'NONE',  ( 10.84999999999990905, 2.500000000000000000, 2.857883832488649301 ) ) ;
#5737=EDGE_LOOP ( 'NONE', ( #17065, #14170 ) ) ;
#5738=PLANE ( 'NONE',  #73227 ) ;
#5739=ORIENTED_EDGE ( 'NONE', *, *, #70059, .F. ) ;
#5740=CARTESIAN_POINT ( 'NONE',  ( 32.28071041562795074, -1.401423001994599904, -4.680142630336261433 ) ) ;
#5741=LINE ( 'NONE', #45702, #72727 ) ;
#5742=FACE_OUTER_BOUND ( 'NONE', #14037, .T. ) ;
#5743=CARTESIAN_POINT ( 'NONE',  ( 19.21290572970625732, -2.587129408759245575, 2.394140119532681688 ) ) ;
#5744=ORIENTED_EDGE ( 'NONE', *, *, #61570, .F. ) ;
#5745=AXIS2_PLACEMENT_3D ( 'NONE', #82970, #122891, #33237 ) ;
#5746=CONICAL_SURFACE ( 'NONE', #22523, 0.1000000000000002554, 0.003490658503988666988 ) ;
#5747=ORIENTED_EDGE ( 'NONE', *, *, #120955, .F. ) ;
#5748=EDGE_LOOP ( 'NONE', ( #32933, #12528, #42354, #100528 ) ) ;
#5749=CARTESIAN_POINT ( 'NONE',  ( -4.600000000000028066, 2.500000000000000000, -3.637306695894650055 ) ) ;
#5750=DIRECTION ( 'NONE',  ( -0.000000000000000000, -1.000000000000000000, -0.000000000000000000 ) ) ;
#5751=CARTESIAN_POINT ( 'NONE',  ( 3.349999999999941913, 2.500000000000000000, 6.395190528383296602 ) ) ;
#5752=FACE_BOUND ( 'NONE', #118185, .T. ) ;
#5753=DIRECTION ( 'NONE',  ( 0.000000000000000000, 1.000000000000000000, 0.000000000000000000 ) ) ;
#5754=DIRECTION ( 'NONE',  ( 0.000000000000000000, 0.000000000000000000, 1.000000000000000000 ) ) ;
#5755=AXIS2_PLACEMENT_3D ( 'NONE', #13640, #72584, #24770 ) ;
#5756=CARTESIAN_POINT ( 'NONE',  ( -0.6000000000000388356, 2.500000000000000000, 3.983716857408420964 ) ) ;
#5757=DIRECTION ( 'NONE',  ( 0.000000000000000000, 1.000000000000000000, 0.000000000000000000 ) ) ;
#5758=CIRCLE ( 'NONE', #118641, 0.06509327318403745899 ) ;
#5759=CIRCLE ( 'NONE', #78962, 0.1000000000000002554 ) ;
#5761=DIRECTION ( 'NONE',  ( 0.000000000000000000, 0.000000000000000000, 1.000000000000000000 ) ) ;
#5762=DIRECTION ( 'NONE',  ( 0.000000000000000000, 1.000000000000000000, 0.000000000000000000 ) ) ;
#5763=AXIS2_PLACEMENT_3D ( 'NONE', #100162, #69395, #71324 ) ;
#5764=EDGE_CURVE ( 'NONE', #69733, #97064, #89562, .T. ) ;
#5765=DIRECTION ( 'NONE',  ( 0.000000000000000000, 0.000000000000000000, 1.000000000000000000 ) ) ;
#5766=EDGE_LOOP ( 'NONE', ( #41133, #58657 ) ) ;
#5767=ORIENTED_EDGE ( 'NONE', *, *, #78247, .T. ) ;
#5768=EDGE_LOOP ( 'NONE', ( #44009, #63234, #75388, #42269 ) ) ;
#5769=VERTEX_POINT ( 'NONE', #92243 ) ;
#5770=CIRCLE ( 'NONE', #18411, 0.06509327318403745899 ) ;
#5771=EDGE_CURVE ( 'NONE', #109919, #15887, #54057, .T. ) ;
#5773=FACE_BOUND ( 'NONE', #29795, .T. ) ;
#5774=EDGE_CURVE ( 'NONE', #41136, #3741, #13022, .T. ) ;
#5775=DIRECTION ( 'NONE',  ( 0.000000000000000000, 0.000000000000000000, 1.000000000000000000 ) ) ;
#5776=CIRCLE ( 'NONE', #78980, 0.09999999999999999167 ) ;
#5777=AXIS2_PLACEMENT_3D ( 'NONE', #57674, #7254, #47210 ) ;
#5778=EDGE_CURVE ( 'NONE', #94129, #52069, #47804, .T. ) ;
#5779=ADVANCED_FACE ( 'NONE', ( #43176 ), #104011, .T. ) ;
#5780=EDGE_LOOP ( 'NONE', ( #117184, #39969 ) ) ;
#5781=CARTESIAN_POINT ( 'NONE',  ( 2.899999999999946620, 2.500000000000000000, -0.5928203230275542746 ) ) ;
#5782=EDGE_CURVE ( 'NONE', #49583, #13385, #118805, .T. ) ;
#5783=DIRECTION ( 'NONE',  ( 0.000000000000000000, 0.000000000000000000, 1.000000000000000000 ) ) ;
#5784=EDGE_CURVE ( 'NONE', #120910, #102673, #5908, .T. ) ;
#5785=AXIS2_PLACEMENT_3D ( 'NONE', #58177, #52207, #124000 ) ;
#5786=VERTEX_POINT ( 'NONE', #3238 ) ;
#5787=CARTESIAN_POINT ( 'NONE',  ( 12.89999999999990088, 12.50000000000000000, -4.330127018922201643 ) ) ;
#5788=CIRCLE ( 'NONE', #49746, 0.1000000000000000472 ) ;
#5789=LINE ( 'NONE', #126229, #38765 ) ;
#5790=AXIS2_PLACEMENT_3D ( 'NONE', #4768, #54522, #125211 ) ;
#5792=DIRECTION ( 'NONE',  ( 0.000000000000000000, 1.000000000000000000, 0.000000000000000000 ) ) ;
#5793=CARTESIAN_POINT ( 'NONE',  ( 8.349999999999923261, 2.500000000000000000, 2.757883832488649656 ) ) ;
#5794=EDGE_CURVE ( 'NONE', #100348, #66863, #94183, .T. ) ;
#5795=CONICAL_SURFACE ( 'NONE', #74784, 0.1000000000000002554, 0.003490658503988666988 ) ;
#5796=AXIS2_PLACEMENT_3D ( 'NONE', #21268, #2263, #73583 ) ;
#5798=AXIS2_PLACEMENT_3D ( 'NONE', #12037, #51985, #112184 ) ;
#5799=DIRECTION ( 'NONE',  ( 0.000000000000000000, 1.000000000000000000, 0.000000000000000000 ) ) ;
#5800=DIRECTION ( 'NONE',  ( 0.000000000000000000, 1.000000000000000000, 0.000000000000000000 ) ) ;
#5801=ORIENTED_EDGE ( 'NONE', *, *, #27504, .F. ) ;
#5802=DIRECTION ( 'NONE',  ( 0.000000000000000000, 0.000000000000000000, -1.000000000000000000 ) ) ;
#5803=ORIENTED_EDGE ( 'NONE', *, *, #91534, .T. ) ;
#5804=ORIENTED_EDGE ( 'NONE', *, *, #24263, .F. ) ;
#5805=VECTOR ( 'NONE', #8255, 1000.000000000000000 ) ;
#5806=CARTESIAN_POINT ( 'NONE',  ( 12.09999999999990550, 12.50000000000000000, 3.637306695894644726 ) ) ;
#5807=ORIENTED_EDGE ( 'NONE', *, *, #27594, .F. ) ;
#5808=DIRECTION ( 'NONE',  ( -0.000000000000000000, -1.000000000000000000, -0.000000000000000000 ) ) ;
#5809=FACE_OUTER_BOUND ( 'NONE', #9872, .T. ) ;
#5810=CIRCLE ( 'NONE', #110294, 0.06509327318403745899 ) ;
#5811=CONICAL_SURFACE ( 'NONE', #60149, 0.09999999999999982514, 0.003490658503988666988 ) ;
#5813=CARTESIAN_POINT ( 'NONE',  ( 10.39999999999991154, 12.50000000000000000, -4.957854068765716882 ) ) ;
#5814=FACE_OUTER_BOUND ( 'NONE', #20646, .T. ) ;
#5815=DIRECTION ( 'NONE',  ( -0.000000000000000000, -1.000000000000000000, -0.000000000000000000 ) ) ;
#5817=DIRECTION ( 'NONE',  ( 0.000000000000000000, 0.000000000000000000, 1.000000000000000000 ) ) ;
#5818=EDGE_CURVE ( 'NONE', #7920, #25044, #123009, .T. ) ;
#5819=CARTESIAN_POINT ( 'NONE',  ( 5.449999999999936229, 2.500000000000000000, 6.495190528383297135 ) ) ;
#5820=DIRECTION ( 'NONE',  ( 0.000000000000000000, 1.000000000000000000, 0.000000000000000000 ) ) ;
#5821=ORIENTED_EDGE ( 'NONE', *, *, #113188, .F. ) ;
#5822=ORIENTED_EDGE ( 'NONE', *, *, #115525, .T. ) ;
#5823=CARTESIAN_POINT ( 'NONE',  ( -9.150000000000009237, 2.500000000000000000, -1.472243186433550122 ) ) ;
#5824=DIRECTION ( 'NONE',  ( 0.000000000000000000, 0.000000000000000000, -1.000000000000000000 ) ) ;
#5825=DIRECTION ( 'NONE',  ( 0.000000000000000000, -0.9999939076577903929, 0.003490651415223739937 ) ) ;
#5826=ORIENTED_EDGE ( 'NONE', *, *, #104827, .F. ) ;
#5827=EDGE_LOOP ( 'NONE', ( #9886, #30996 ) ) ;
#5828=ORIENTED_EDGE ( 'NONE', *, *, #26699, .T. ) ;
#5829=EDGE_CURVE ( 'NONE', #37944, #92178, #85002, .T. ) ;
#5830=DIRECTION ( 'NONE',  ( -0.000000000000000000, 1.000000000000000000, -0.000000000000000000 ) ) ;
#5831=EDGE_CURVE ( 'NONE', #72089, #54959, #121044, .T. ) ;
#5832=CARTESIAN_POINT ( 'NONE',  ( -6.650000000000014566, 2.500000000000000000, 6.495190528383297135 ) ) ;
#5833=DIRECTION ( 'NONE',  ( -0.000000000000000000, 1.000000000000000000, -0.000000000000000000 ) ) ;
#5834=EDGE_CURVE ( 'NONE', #114185, #2568, #62803, .T. ) ;
#5836=DIRECTION ( 'NONE',  ( -0.000000000000000000, 1.000000000000000000, -0.000000000000000000 ) ) ;
#5837=DIRECTION ( 'NONE',  ( -4.274815082592931898E-19, -0.9999939076577903929, -0.003490651415223739937 ) ) ;
#5838=DIRECTION ( 'NONE',  ( -0.000000000000000000, -1.000000000000000000, -0.000000000000000000 ) ) ;
#5839=DIRECTION ( 'NONE',  ( -0.000000000000000000, -1.000000000000000000, -0.000000000000000000 ) ) ;
#5840=DIRECTION ( 'NONE',  ( 0.000000000000000000, 0.000000000000000000, 1.000000000000000000 ) ) ;
#5841=EDGE_CURVE ( 'NONE', #51535, #126108, #35290, .T. ) ;
#5842=DIRECTION ( 'NONE',  ( 0.000000000000000000, 1.000000000000000000, 0.000000000000000000 ) ) ;
#5843=EDGE_CURVE ( 'NONE', #40852, #3310, #123630, .T. ) ;
#5844=EDGE_CURVE ( 'NONE', #71057, #115877, #6017, .T. ) ;
#5845=EDGE_LOOP ( 'NONE', ( #90256, #16620 ) ) ;
#5846=CONICAL_SURFACE ( 'NONE', #28861, 0.1000000000000002554, 0.003490658503988666988 ) ;
#5847=ADVANCED_FACE ( 'NONE', ( #24806 ), #64719, .T. ) ;
#5848=FACE_OUTER_BOUND ( 'NONE', #60487, .T. ) ;
#5849=ORIENTED_EDGE ( 'NONE', *, *, #2862, .T. ) ;
#5850=EDGE_LOOP ( 'NONE', ( #24162, #77212 ) ) ;
#5851=CARTESIAN_POINT ( 'NONE',  ( 0.3999999999999628852, 12.50000000000000000, -0.6928203230275520319 ) ) ;
#5852=FACE_OUTER_BOUND ( 'NONE', #14068, .T. ) ;
#5853=CARTESIAN_POINT ( 'NONE',  ( -10.40000000000000213, 2.500000000000000000, -5.022947341949749678 ) ) ;
#5854=ADVANCED_FACE ( 'NONE', ( #5150 ), #45101, .T. ) ;
#5855=CIRCLE ( 'NONE', #72689, 0.06509327318403745899 ) ;
#5856=CARTESIAN_POINT ( 'NONE',  ( -0.6000000000000383915, 12.50000000000000000, -3.983716857408426293 ) ) ;
#5857=CIRCLE ( 'NONE', #41505, 0.1000000000000000472 ) ;
#5858=DIRECTION ( 'NONE',  ( -4.274815082592931898E-19, -0.9999939076577903929, -0.003490651415223739937 ) ) ;
#5859=DIRECTION ( 'NONE',  ( 0.000000000000000000, 0.000000000000000000, -1.000000000000000000 ) ) ;
#5860=LINE ( 'NONE', #37287, #90646 ) ;
#5861=ORIENTED_EDGE ( 'NONE', *, *, #86570, .F. ) ;
#5862=DIRECTION ( 'NONE',  ( -4.274815082592931898E-19, -0.9999939076577903929, -0.003490651415223739937 ) ) ;
#5863=LINE ( 'NONE', #53695, #83327 ) ;
#5864=EDGE_LOOP ( 'NONE', ( #42066, #121420 ) ) ;
#5865=CONICAL_SURFACE ( 'NONE', #1754, 0.1000000000000000056, 0.003490658503988666988 ) ;
#5866=ORIENTED_EDGE ( 'NONE', *, *, #110867, .T. ) ;
#5867=VERTEX_POINT ( 'NONE', #85653 ) ;
#5868=CIRCLE ( 'NONE', #8021, 0.1000000000000002554 ) ;
#5869=EDGE_LOOP ( 'NONE', ( #125294, #13998, #10454, #106543 ) ) ;
#5870=CARTESIAN_POINT ( 'NONE',  ( -3.550000000000030909, 12.50000000000000000, -6.841600689897078702 ) ) ;
#5871=DIRECTION ( 'NONE',  ( -0.000000000000000000, 1.000000000000000000, -0.000000000000000000 ) ) ;
#5872=CONICAL_SURFACE ( 'NONE', #102138, 0.09999999999999982514, 0.003490658503988666988 ) ;
#5873=CARTESIAN_POINT ( 'NONE',  ( 9.599999999999914380, 2.500000000000000000, -3.637306695894650055 ) ) ;
#5874=LINE ( 'NONE', #5242, #2686 ) ;
#5875=CARTESIAN_POINT ( 'NONE',  ( 9.999999999999911182, 12.50000000000000000, 5.088040615133786027 ) ) ;
#5876=EDGE_LOOP ( 'NONE', ( #10322, #116225 ) ) ;
#5877=DIRECTION ( 'NONE',  ( -4.274815082592931898E-19, -0.9999939076577903929, -0.003490651415223739937 ) ) ;
#5878=CIRCLE ( 'NONE', #22647, 0.1000000000000002554 ) ;
#5879=CONICAL_SURFACE ( 'NONE', #79079, 0.09999999999999982514, 0.003490658503988666988 ) ;
#5880=LINE ( 'NONE', #85741, #22786 ) ;
#5881=ORIENTED_EDGE ( 'NONE', *, *, #88282, .T. ) ;
#5882=AXIS2_PLACEMENT_3D ( 'NONE', #92358, #2680, #19773 ) ;
#5883=EDGE_CURVE ( 'NONE', #66538, #119116, #3967, .T. ) ;
#5884=VERTEX_POINT ( 'NONE', #117021 ) ;
#5885=ORIENTED_EDGE ( 'NONE', *, *, #91262, .T. ) ;
#5886=DIRECTION ( 'NONE',  ( -0.000000000000000000, -1.000000000000000000, -0.000000000000000000 ) ) ;
#5887=DIRECTION ( 'NONE',  ( 0.000000000000000000, 0.000000000000000000, 1.000000000000000000 ) ) ;
#5888=DIRECTION ( 'NONE',  ( 0.000000000000000000, 1.000000000000000000, 0.000000000000000000 ) ) ;
#5889=EDGE_LOOP ( 'NONE', ( #37233, #106184, #50325, #128711 ) ) ;
#5890=CARTESIAN_POINT ( 'NONE',  ( 4.999999999999936939, 2.500000000000000000, -3.637306695894650055 ) ) ;
#5892=EDGE_CURVE ( 'NONE', #87369, #41701, #31189, .T. ) ;
#5893=DIRECTION ( 'NONE',  ( 0.000000000000000000, -0.9999939076577903929, 0.003490651415223739937 ) ) ;
#5894=DIRECTION ( 'NONE',  ( -0.000000000000000000, 1.000000000000000000, -0.000000000000000000 ) ) ;
#5895=DIRECTION ( 'NONE',  ( 0.000000000000000000, 0.000000000000000000, 1.000000000000000000 ) ) ;
#5896=EDGE_LOOP ( 'NONE', ( #122123, #125014 ) ) ;
#5897=CIRCLE ( 'NONE', #118788, 0.1000000000000002554 ) ;
#5898=CONICAL_SURFACE ( 'NONE', #43508, 0.1000000000000002554, 0.003490658503988666988 ) ;
#5899=DIRECTION ( 'NONE',  ( 0.000000000000000000, 0.000000000000000000, 1.000000000000000000 ) ) ;
#5900=ORIENTED_EDGE ( 'NONE', *, *, #22942, .T. ) ;
#5901=ORIENTED_EDGE ( 'NONE', *, *, #56326, .T. ) ;
#5902=ORIENTED_EDGE ( 'NONE', *, *, #72453, .T. ) ;
#5903=DIRECTION ( 'NONE',  ( 0.000000000000000000, 1.000000000000000000, 0.000000000000000000 ) ) ;
#5904=FACE_BOUND ( 'NONE', #67365, .T. ) ;
#5906=DIRECTION ( 'NONE',  ( -0.000000000000000000, -1.000000000000000000, -0.000000000000000000 ) ) ;
#5907=DIRECTION ( 'NONE',  ( -0.000000000000000000, -1.000000000000000000, -0.000000000000000000 ) ) ;
#5908=CIRCLE ( 'NONE', #49875, 0.1000000000000000056 ) ;
#5909=ORIENTED_EDGE ( 'NONE', *, *, #69506, .F. ) ;
#5910=DIRECTION ( 'NONE',  ( 0.000000000000000000, 0.000000000000000000, 1.000000000000000000 ) ) ;
#5911=LINE ( 'NONE', #115887, #26015 ) ;
#5912=FACE_OUTER_BOUND ( 'NONE', #73383, .T. ) ;
#5913=DIRECTION ( 'NONE',  ( 0.000000000000000000, 1.000000000000000000, 0.000000000000000000 ) ) ;
#5914=ORIENTED_EDGE ( 'NONE', *, *, #51214, .F. ) ;
#5915=DIRECTION ( 'NONE',  ( 0.000000000000000000, 0.000000000000000000, -1.000000000000000000 ) ) ;
#5916=AXIS2_PLACEMENT_3D ( 'NONE', #117936, #58400, #18455 ) ;
#5917=ADVANCED_FACE ( 'NONE', ( #67260 ), #66651, .T. ) ;
#5918=AXIS2_PLACEMENT_3D ( 'NONE', #60628, #30529, #21318 ) ;
#5919=DIRECTION ( 'NONE',  ( 0.000000000000000000, 0.000000000000000000, 1.000000000000000000 ) ) ;
#5920=CIRCLE ( 'NONE', #37548, 0.06509327318403745899 ) ;
#5921=ORIENTED_EDGE ( 'NONE', *, *, #120359, .T. ) ;
#5922=CARTESIAN_POINT ( 'NONE',  ( 5.199999999999933564, 12.50000000000000000, 0.3464101615137735735 ) ) ;
#5923=FACE_BOUND ( 'NONE', #119940, .T. ) ;
#5924=EDGE_CURVE ( 'NONE', #50242, #59628, #116391, .T. ) ;
#5925=DIRECTION ( 'NONE',  ( 0.000000000000000000, 0.000000000000000000, 1.000000000000000000 ) ) ;
#5926=AXIS2_PLACEMENT_3D ( 'NONE', #58007, #98537, #128705 ) ;
#5927=CONICAL_SURFACE ( 'NONE', #47733, 0.1000000000000002554, 0.003490658503988666988 ) ;
#5928=VECTOR ( 'NONE', #83825, 1000.000000000000000 ) ;
#5929=ORIENTED_EDGE ( 'NONE', *, *, #87428, .F. ) ;
#5930=DIRECTION ( 'NONE',  ( -0.000000000000000000, -1.000000000000000000, -0.000000000000000000 ) ) ;
#5931=FACE_OUTER_BOUND ( 'NONE', #19012, .T. ) ;
#5932=EDGE_CURVE ( 'NONE', #27373, #69211, #74985, .T. ) ;
#5933=ORIENTED_EDGE ( 'NONE', *, *, #44218, .F. ) ;
#5934=EDGE_CURVE ( 'NONE', #121533, #10045, #37443, .T. ) ;
#5935=ORIENTED_EDGE ( 'NONE', *, *, #106790, .T. ) ;
#5936=ADVANCED_FACE ( 'NONE', ( #128168 ), #64609, .T. ) ;
#5937=EDGE_CURVE ( 'NONE', #74378, #124598, #47905, .T. ) ;
#5939=ADVANCED_FACE ( 'NONE', ( #126878 ), #110580, .T. ) ;
#5940=VECTOR ( 'NONE', #83697, 1000.000000000000000 ) ;
#5941=ORIENTED_EDGE ( 'NONE', *, *, #55971, .F. ) ;
#5943=FACE_OUTER_BOUND ( 'NONE', #39851, .T. ) ;
#5944=DIRECTION ( 'NONE',  ( 0.000000000000000000, 0.000000000000000000, 1.000000000000000000 ) ) ;
#5945=CARTESIAN_POINT ( 'NONE',  ( 2.299999999999948752, 2.500000000000000000, 0.3464101615137735735 ) ) ;
#5946=CARTESIAN_POINT ( 'NONE',  ( -0.4000000000000401013, 12.50000000000000000, -3.572213422710612374 ) ) ;
#5947=EDGE_CURVE ( 'NONE', #3753, #72399, #39513, .T. ) ;
#5948=EDGE_CURVE ( 'NONE', #44658, #72823, #37839, .T. ) ;
#5949=AXIS2_PLACEMENT_3D ( 'NONE', #79088, #29346, #109826 ) ;
#5950=EDGE_CURVE ( 'NONE', #120001, #39091, #20709, .T. ) ;
#5951=EDGE_LOOP ( 'NONE', ( #116376, #78578 ) ) ;
#5952=EDGE_LOOP ( 'NONE', ( #78835, #1359 ) ) ;
#5953=CARTESIAN_POINT ( 'NONE',  ( -4.200000000000025935, 12.50000000000000000, 0.06509327318403504425 ) ) ;
#5954=FACE_OUTER_BOUND ( 'NONE', #120034, .T. ) ;
#5955=CIRCLE ( 'NONE', #16406, 0.1000000000000002554 ) ;
#5956=DIRECTION ( 'NONE',  ( -0.000000000000000000, 1.000000000000000000, -0.000000000000000000 ) ) ;
#5957=CONICAL_SURFACE ( 'NONE', #110434, 0.1000000000000002554, 0.003490658503988666988 ) ;
#5958=DIRECTION ( 'NONE',  ( -0.000000000000000000, -1.000000000000000000, -0.000000000000000000 ) ) ;
#5959=EDGE_LOOP ( 'NONE', ( #80506, #11905 ) ) ;
#5960=ORIENTED_EDGE ( 'NONE', *, *, #95414, .T. ) ;
#5961=DIRECTION ( 'NONE',  ( 0.000000000000000000, -0.000000000000000000, -1.000000000000000000 ) ) ;
#5962=ORIENTED_EDGE ( 'NONE', *, *, #39520, .T. ) ;
#5963=DIRECTION ( 'NONE',  ( -0.000000000000000000, -1.000000000000000000, -0.000000000000000000 ) ) ;
#5965=ORIENTED_EDGE ( 'NONE', *, *, #79151, .T. ) ;
#5966=DIRECTION ( 'NONE',  ( 0.000000000000000000, -0.000000000000000000, 1.000000000000000000 ) ) ;
#5967=AXIS2_PLACEMENT_3D ( 'NONE', #113759, #24086, #64005 ) ;
#5968=DIRECTION ( 'NONE',  ( 0.000000000000000000, -0.9999939076577903929, 0.003490651415223739937 ) ) ;
#5969=CARTESIAN_POINT ( 'NONE',  ( 6.449999999999933564, 2.500000000000000000, -6.941600689897078347 ) ) ;
#5970=DIRECTION ( 'NONE',  ( 0.000000000000000000, 1.000000000000000000, 0.000000000000000000 ) ) ;
#5972=DIRECTION ( 'NONE',  ( 0.000000000000000000, -0.9999939076577903929, 0.003490651415223739937 ) ) ;
#5973=CARTESIAN_POINT ( 'NONE',  ( -9.800000000000004263, 2.500000000000000000, 3.983716857408420076 ) ) ;
#5976=VECTOR ( 'NONE', #32457, 1000.000000000000000 ) ;
#5977=CARTESIAN_POINT ( 'NONE',  ( -1.250000000000037526, 2.500000000000000000, -5.802370205355749988 ) ) ;
#5978=VERTEX_POINT ( 'NONE', #96113 ) ;
#5979=ORIENTED_EDGE ( 'NONE', *, *, #93620, .T. ) ;
#5980=CARTESIAN_POINT ( 'NONE',  ( 9.999999999999911182, 12.50000000000000000, 4.957854068765711553 ) ) ;
#5981=ORIENTED_EDGE ( 'NONE', *, *, #9236, .F. ) ;
#5982=DIRECTION ( 'NONE',  ( 0.000000000000000000, 1.000000000000000000, 0.000000000000000000 ) ) ;
#5983=ADVANCED_FACE ( 'NONE', ( #6413 ), #12276, .T. ) ;
#5984=ORIENTED_EDGE ( 'NONE', *, *, #100999, .F. ) ;
#5985=VERTEX_POINT ( 'NONE', #86279 ) ;
#5986=ORIENTED_EDGE ( 'NONE', *, *, #41795, .T. ) ;
#5987=AXIS2_PLACEMENT_3D ( 'NONE', #9363, #19837, #49313 ) ;
#5988=DIRECTION ( 'NONE',  ( 0.000000000000000000, 0.000000000000000000, 1.000000000000000000 ) ) ;
#5989=CARTESIAN_POINT ( 'NONE',  ( -6.650000000000014566, 2.500000000000000000, 5.802370205355744659 ) ) ;
#5991=AXIS2_PLACEMENT_3D ( 'NONE', #35402, #36044, #102825 ) ;
#5992=CARTESIAN_POINT ( 'NONE',  ( 7.899999999999924860, 12.50000000000000000, -5.022947341949754119 ) ) ;
#5993=DIRECTION ( 'NONE',  ( 0.000000000000000000, 1.000000000000000000, 0.000000000000000000 ) ) ;
#5994=DIRECTION ( 'NONE',  ( 0.000000000000000000, 1.000000000000000000, 0.000000000000000000 ) ) ;
#5995=CIRCLE ( 'NONE', #118885, 0.09999999999999982514 ) ;
#5996=ORIENTED_EDGE ( 'NONE', *, *, #12308, .F. ) ;
#5998=DIRECTION ( 'NONE',  ( -4.274815082592931898E-19, -0.9999939076577903929, -0.003490651415223739937 ) ) ;
#5999=ORIENTED_EDGE ( 'NONE', *, *, #913, .T. ) ;
#6000=ADVANCED_FACE ( 'NONE', ( #7072 ), #114775, .T. ) ;
#6001=AXIS2_PLACEMENT_3D ( 'NONE', #44783, #43497, #34327 ) ;
#6002=AXIS2_PLACEMENT_3D ( 'NONE', #73853, #24116, #64038 ) ;
#6003=ORIENTED_EDGE ( 'NONE', *, *, #61264, .T. ) ;
#6004=ORIENTED_EDGE ( 'NONE', *, *, #97858, .T. ) ;
#6005=ORIENTED_EDGE ( 'NONE', *, *, #97270, .F. ) ;
#6006=ADVANCED_FACE ( 'NONE', ( #58142 ), #26970, .T. ) ;
#6008=ORIENTED_EDGE ( 'NONE', *, *, #72780, .T. ) ;
#6009=ORIENTED_EDGE ( 'NONE', *, *, #54720, .F. ) ;
#6010=PLANE ( 'NONE',  #115515 ) ;
#6011=EDGE_CURVE ( 'NONE', #100878, #84422, #127316, .T. ) ;
#6012=FACE_OUTER_BOUND ( 'NONE', #70877, .T. ) ;
#6013=DIRECTION ( 'NONE',  ( 0.000000000000000000, 0.000000000000000000, -1.000000000000000000 ) ) ;
#6014=DIRECTION ( 'NONE',  ( 0.000000000000000000, 1.000000000000000000, 0.000000000000000000 ) ) ;
#6015=DIRECTION ( 'NONE',  ( -0.000000000000000000, -1.000000000000000000, -0.000000000000000000 ) ) ;
#6016=CARTESIAN_POINT ( 'NONE',  ( 3.549999999999944755, 12.50000000000000000, -2.511473670974877948 ) ) ;
#6017=CIRCLE ( 'NONE', #125168, 0.06509327318403745899 ) ;
#6018=ORIENTED_EDGE ( 'NONE', *, *, #95348, .F. ) ;
#6019=DIRECTION ( 'NONE',  ( 0.000000000000000000, 1.000000000000000000, 0.000000000000000000 ) ) ;
#6020=ORIENTED_EDGE ( 'NONE', *, *, #94886, .F. ) ;
#6021=CIRCLE ( 'NONE', #39519, 0.1000000000000000472 ) ;
#6022=DIRECTION ( 'NONE',  ( 0.000000000000000000, 1.000000000000000000, 0.000000000000000000 ) ) ;
#6024=EDGE_LOOP ( 'NONE', ( #21122, #73375 ) ) ;
#6025=CARTESIAN_POINT ( 'NONE',  ( 14.59999999999989484, 12.50000000000000000, -2.276824562219559311E-15 ) ) ;
#6027=ORIENTED_EDGE ( 'NONE', *, *, #36244, .F. ) ;
#6028=EDGE_CURVE ( 'NONE', #39107, #18925, #118983, .T. ) ;
#6029=VERTEX_POINT ( 'NONE', #21927 ) ;
#6030=CARTESIAN_POINT ( 'NONE',  ( 9.149999999999916866, 12.50000000000000000, 7.188010851410848723 ) ) ;
#6031=AXIS2_PLACEMENT_3D ( 'NONE', #67700, #118093, #105043 ) ;
#6032=DIRECTION ( 'NONE',  ( 0.000000000000000000, 1.000000000000000000, 0.000000000000000000 ) ) ;
#6033=VECTOR ( 'NONE', #18893, 1000.000000000000000 ) ;
#6034=DIRECTION ( 'NONE',  ( 0.000000000000000000, 0.000000000000000000, 1.000000000000000000 ) ) ;
#6035=DIRECTION ( 'NONE',  ( 0.000000000000000000, 0.000000000000000000, 1.000000000000000000 ) ) ;
#6036=LINE ( 'NONE', #84618, #67933 ) ;
#6037=VERTEX_POINT ( 'NONE', #121397 ) ;
#6038=DIRECTION ( 'NONE',  ( 0.000000000000000000, 0.000000000000000000, -1.000000000000000000 ) ) ;
#6039=FACE_OUTER_BOUND ( 'NONE', #24073, .T. ) ;
#6040=FACE_OUTER_BOUND ( 'NONE', #15763, .T. ) ;
#6041=DIRECTION ( 'NONE',  ( 0.000000000000000000, 1.000000000000000000, 0.000000000000000000 ) ) ;
#6042=DIRECTION ( 'NONE',  ( 0.000000000000000000, 0.000000000000000000, 1.000000000000000000 ) ) ;
#6043=CIRCLE ( 'NONE', #22809, 0.09999999999999999167 ) ;
#6044=EDGE_LOOP ( 'NONE', ( #38454, #21595 ) ) ;
#6045=EDGE_CURVE ( 'NONE', #59553, #49236, #83407, .T. ) ;
#6046=ORIENTED_EDGE ( 'NONE', *, *, #61421, .F. ) ;
#6048=ORIENTED_EDGE ( 'NONE', *, *, #13327, .F. ) ;
#6049=DIRECTION ( 'NONE',  ( 0.000000000000000000, 0.000000000000000000, -1.000000000000000000 ) ) ;
#6050=DIRECTION ( 'NONE',  ( -0.000000000000000000, 1.000000000000000000, -0.000000000000000000 ) ) ;
#6051=AXIS2_PLACEMENT_3D ( 'NONE', #2424, #74902, #116105 ) ;
#6052=AXIS2_PLACEMENT_3D ( 'NONE', #61614, #41966, #81865 ) ;
#6054=DIRECTION ( 'NONE',  ( -0.000000000000000000, -1.000000000000000000, -0.000000000000000000 ) ) ;
#6055=DIRECTION ( 'NONE',  ( 0.000000000000000000, 0.000000000000000000, -1.000000000000000000 ) ) ;
#6056=EDGE_CURVE ( 'NONE', #82618, #121714, #118902, .T. ) ;
#6058=DIRECTION ( 'NONE',  ( -0.000000000000000000, -1.000000000000000000, -0.000000000000000000 ) ) ;
#6059=ORIENTED_EDGE ( 'NONE', *, *, #115171, .F. ) ;
#6060=CARTESIAN_POINT ( 'NONE',  ( -3.350000000000028511, 2.500000000000000000, -1.372243186433550033 ) ) ;
#6061=DIRECTION ( 'NONE',  ( 0.000000000000000000, 0.000000000000000000, -1.000000000000000000 ) ) ;
#6062=CIRCLE ( 'NONE', #123155, 0.09999999999999982514 ) ;
#6063=EDGE_LOOP ( 'NONE', ( #4227, #7198, #72515, #3551 ) ) ;
#6064=ADVANCED_FACE ( 'NONE', ( #31735 ), #51395, .T. ) ;
#6065=DIRECTION ( 'NONE',  ( 0.000000000000000000, 0.000000000000000000, 1.000000000000000000 ) ) ;
#6066=AXIS2_PLACEMENT_3D ( 'NONE', #84743, #24536, #14048 ) ;
#6067=DIRECTION ( 'NONE',  ( 0.000000000000000000, 1.000000000000000000, 0.000000000000000000 ) ) ;
#6068=CARTESIAN_POINT ( 'NONE',  ( -1.250000000000036193, 2.500000000000000000, 5.802370205355744659 ) ) ;
#6069=VECTOR ( 'NONE', #55985, 1000.000000000000000 ) ;
#6070=ORIENTED_EDGE ( 'NONE', *, *, #90083, .F. ) ;
#6071=DIRECTION ( 'NONE',  ( 0.000000000000000000, 0.000000000000000000, 1.000000000000000000 ) ) ;
#6072=VERTEX_POINT ( 'NONE', #71656 ) ;
#6073=CARTESIAN_POINT ( 'NONE',  ( 3.749999999999978684, 2.500000000000000000, -6.495190528383302464 ) ) ;
#6074=CONICAL_SURFACE ( 'NONE', #87558, 0.1000000000000002554, 0.003490658503988666988 ) ;
#6075=DIRECTION ( 'NONE',  ( 0.000000000000000000, 0.000000000000000000, 1.000000000000000000 ) ) ;
#6076=ORIENTED_EDGE ( 'NONE', *, *, #33309, .F. ) ;
#6077=CARTESIAN_POINT ( 'NONE',  ( 4.399999999999940847, 2.500000000000000000, -3.983716857408426293 ) ) ;
#6079=CIRCLE ( 'NONE', #93839, 0.06509327318403745899 ) ;
#6080=DIRECTION ( 'NONE',  ( -0.000000000000000000, 1.000000000000000000, -0.000000000000000000 ) ) ;
#6081=ORIENTED_EDGE ( 'NONE', *, *, #22010, .T. ) ;
#6082=ORIENTED_EDGE ( 'NONE', *, *, #95191, .F. ) ;
#6083=PLANE ( 'NONE',  #111985 ) ;
#6084=EDGE_CURVE ( 'NONE', #128192, #90718, #58779, .T. ) ;
#6085=AXIS2_PLACEMENT_3D ( 'NONE', #12940, #52891, #33890 ) ;
#6086=AXIS2_PLACEMENT_3D ( 'NONE', #12182, #63237, #2351 ) ;
#6087=ORIENTED_EDGE ( 'NONE', *, *, #61244, .T. ) ;
#6088=FACE_OUTER_BOUND ( 'NONE', #72111, .T. ) ;
#6089=CARTESIAN_POINT ( 'NONE',  ( -12.49999999999995737, 2.500000000000000000, 4.430127018922196847 ) ) ;
#6090=EDGE_CURVE ( 'NONE', #124494, #42905, #89657, .T. ) ;
#6091=ADVANCED_FACE ( 'NONE', ( #72949 ), #100124, .T. ) ;
#6092=ORIENTED_EDGE ( 'NONE', *, *, #60713, .T. ) ;
#6093=ADVANCED_FACE ( 'NONE', ( #29325 ), #85540, .T. ) ;
#6094=ADVANCED_FACE ( 'NONE', ( #23191 ), #109146, .T. ) ;
#6095=CARTESIAN_POINT ( 'NONE',  ( 7.949999999999925571, 2.500000000000000000, -6.495190528383302464 ) ) ;
#6096=CARTESIAN_POINT ( 'NONE',  ( -13.94999999999998685, 12.50000000000000000, -2.511473670974875727 ) ) ;
#6097=EDGE_LOOP ( 'NONE', ( #10210, #87511 ) ) ;
#6098=CARTESIAN_POINT ( 'NONE',  ( -3.550000000000028244, 12.50000000000000000, 2.511473670974873507 ) ) ;
#6099=CARTESIAN_POINT ( 'NONE',  ( 8.549999999999922551, 2.500000000000000000, -6.048780366869526581 ) ) ;
#6100=ADVANCED_FACE ( 'NONE', ( #53319 ), #102413, .T. ) ;
#6101=CARTESIAN_POINT ( 'NONE',  ( 16.56576425165007649, -1.499999999999997113, -6.084390597445788806 ) ) ;
#6102=CIRCLE ( 'NONE', #73024, 0.1000000000000000056 ) ;
#6103=FACE_OUTER_BOUND ( 'NONE', #52348, .T. ) ;
#6104=ADVANCED_FACE ( 'NONE', ( #82121 ), #83422, .T. ) ;
#6105=CARTESIAN_POINT ( 'NONE',  ( -8.350000000000013856, 2.500000000000000000, 2.165063509461097713 ) ) ;
#6106=CARTESIAN_POINT ( 'NONE',  ( -7.900000000000011013, 2.500000000000000000, 5.122947341949749323 ) ) ;
#6107=EDGE_CURVE ( 'NONE', #50779, #62968, #114869, .T. ) ;
#6108=ADVANCED_FACE ( 'NONE', ( #33044 ), #41576, .T. ) ;
#6109=VECTOR ( 'NONE', #94127, 1000.000000000000000 ) ;
#6110=ADVANCED_FACE ( 'NONE', ( #18840 ), #47992, .T. ) ;
#6111=AXIS2_PLACEMENT_3D ( 'NONE', #49053, #88959, #78514 ) ;
#6112=ORIENTED_EDGE ( 'NONE', *, *, #39836, .F. ) ;
#6113=EDGE_LOOP ( 'NONE', ( #71080, #14286 ) ) ;
#6114=EDGE_LOOP ( 'NONE', ( #47227, #23549 ) ) ;
#6115=ORIENTED_EDGE ( 'NONE', *, *, #108452, .F. ) ;
#6116=CARTESIAN_POINT ( 'NONE',  ( 65.38811649227257305, 3.824344232458577242, 5.305600839591995133 ) ) ;
#6117=DIRECTION ( 'NONE',  ( 0.000000000000000000, -0.9999939076577903929, 0.003490651415223739937 ) ) ;
#6118=DIRECTION ( 'NONE',  ( 0.000000000000000000, 0.000000000000000000, 1.000000000000000000 ) ) ;
#6119=ORIENTED_EDGE ( 'NONE', *, *, #56735, .F. ) ;
#6120=FACE_BOUND ( 'NONE', #53041, .T. ) ;
#6121=EDGE_CURVE ( 'NONE', #8342, #49328, #86625, .T. ) ;
#6122=CARTESIAN_POINT ( 'NONE',  ( 10.64999999999991331, 2.500000000000000000, 6.148780366869520897 ) ) ;
#6123=DIRECTION ( 'NONE',  ( 0.000000000000000000, 1.000000000000000000, 0.000000000000000000 ) ) ;
#6124=CIRCLE ( 'NONE', #116933, 0.06509327318403745899 ) ;
#6125=FACE_OUTER_BOUND ( 'NONE', #105982, .T. ) ;
#6126=CIRCLE ( 'NONE', #79320, 0.06509327318403745899 ) ;
#6127=CARTESIAN_POINT ( 'NONE',  ( -10.45000000000000107, 2.500000000000000000, 6.395190528383296602 ) ) ;
#6128=LINE ( 'NONE', #46076, #99421 ) ;
#6129=DIRECTION ( 'NONE',  ( 0.000000000000000000, 0.000000000000000000, 1.000000000000000000 ) ) ;
#6130=CARTESIAN_POINT ( 'NONE',  ( -2.499999999999996003, 12.50000000000000000, -4.395220292106239768 ) ) ;
#6131=FACE_OUTER_BOUND ( 'NONE', #32652, .T. ) ;
#6132=CARTESIAN_POINT ( 'NONE',  ( -2.300000000000032685, 2.500000000000000000, -4.776537180435978414 ) ) ;
#6133=AXIS2_PLACEMENT_3D ( 'NONE', #35582, #83393, #75482 ) ;
#6134=DIRECTION ( 'NONE',  ( 0.000000000000000000, -0.9999939076577903929, 0.003490651415223739937 ) ) ;
#6135=CIRCLE ( 'NONE', #96036, 0.06509327318403745899 ) ;
#6136=ORIENTED_EDGE ( 'NONE', *, *, #127672, .F. ) ;
#6137=EDGE_LOOP ( 'NONE', ( #25763, #44126, #111832, #122322 ) ) ;
#6138=CONICAL_SURFACE ( 'NONE', #89773, 0.1000000000000000472, 0.003490658503988666988 ) ;
#6139=ORIENTED_EDGE ( 'NONE', *, *, #40240, .F. ) ;
#6140=EDGE_LOOP ( 'NONE', ( #21883, #123981, #5088, #4039 ) ) ;
#6141=DIRECTION ( 'NONE',  ( -4.274815082592931898E-19, -0.9999939076577903929, -0.003490651415223739937 ) ) ;
#6142=ORIENTED_EDGE ( 'NONE', *, *, #36245, .F. ) ;
#6143=DIRECTION ( 'NONE',  ( 0.000000000000000000, 0.000000000000000000, -1.000000000000000000 ) ) ;
#6144=ORIENTED_EDGE ( 'NONE', *, *, #24897, .T. ) ;
#6145=VERTEX_POINT ( 'NONE', #93877 ) ;
#6146=CARTESIAN_POINT ( 'NONE',  ( 7.699999999999923794, 12.50000000000000000, -0.4115034346978157509 ) ) ;
#6147=PRODUCT_DEFINITION_CONTEXT ( 'detailed design', #84818, 'design' ) ;
#6148=CARTESIAN_POINT ( 'NONE',  ( 7.180215335588899350, -2.499999999999999556, 8.697219394723605390 ) ) ;
#6149=DIRECTION ( 'NONE',  ( 0.000000000000000000, 0.000000000000000000, -1.000000000000000000 ) ) ;
#6150=LINE ( 'NONE', #27100, #3281 ) ;
#6151=CARTESIAN_POINT ( 'NONE',  ( -4.999999999999990230, 12.50000000000000000, -4.265033745738164406 ) ) ;
#6153=ORIENTED_EDGE ( 'NONE', *, *, #122112, .F. ) ;
#6154=ADVANCED_FACE ( 'NONE', ( #53954 ), #64409, .T. ) ;
#6155=VERTEX_POINT ( 'NONE', #44128 ) ;
#6156=VERTEX_POINT ( 'NONE', #73572 ) ;
#6157=EDGE_CURVE ( 'NONE', #1899, #106239, #65697, .T. ) ;
#6159=ORIENTED_EDGE ( 'NONE', *, *, #49847, .T. ) ;
#6160=ORIENTED_EDGE ( 'NONE', *, *, #105601, .F. ) ;
#6161=CIRCLE ( 'NONE', #79350, 0.1000000000000002554 ) ;
#6162=DIRECTION ( 'NONE',  ( -0.000000000000000000, -1.000000000000000000, -0.000000000000000000 ) ) ;
#6163=ADVANCED_FACE ( 'NONE', ( #15935 ), #20795, .T. ) ;
#6164=CARTESIAN_POINT ( 'NONE',  ( -0.4000000000000392131, 2.500000000000000000, -5.022947341949754119 ) ) ;
#6165=CARTESIAN_POINT ( 'NONE',  ( 12.29999999999990479, 12.50000000000000000, -3.983716857408426293 ) ) ;
#6166=DIRECTION ( 'NONE',  ( 0.000000000000000000, 0.000000000000000000, -1.000000000000000000 ) ) ;
#6167=FACE_OUTER_BOUND ( 'NONE', #74923, .T. ) ;
#6168=CARTESIAN_POINT ( 'NONE',  ( -2.700000000000029932, 12.50000000000000000, -4.676537180435977881 ) ) ;
#6169=CONICAL_SURFACE ( 'NONE', #79358, 0.1000000000000002554, 0.003490658503988666988 ) ;
#6170=EDGE_LOOP ( 'NONE', ( #32732, #28435, #114957, #112577 ) ) ;
#6171=LINE ( 'NONE', #86013, #1025 ) ;
#6172=ORIENTED_EDGE ( 'NONE', *, *, #3997, .T. ) ;
#6173=DIRECTION ( 'NONE',  ( 0.000000000000000000, 0.000000000000000000, 1.000000000000000000 ) ) ;
#6174=AXIS2_PLACEMENT_3D ( 'NONE', #82215, #30558, #71102 ) ;
#6175=AXIS2_PLACEMENT_3D ( 'NONE', #90120, #119590, #49594 ) ;
#6177=CARTESIAN_POINT ( 'NONE',  ( 5.449999999999937117, 2.500000000000000000, -6.395190528383301931 ) ) ;
#6178=FACE_OUTER_BOUND ( 'NONE', #115819, .T. ) ;
#6179=ORIENTED_EDGE ( 'NONE', *, *, #12622, .F. ) ;
#6180=AXIS2_PLACEMENT_3D ( 'NONE', #2254, #22583, #73573 ) ;
#6181=FACE_OUTER_BOUND ( 'NONE', #28408, .T. ) ;
#6182=DIRECTION ( 'NONE',  ( -4.274815082592931898E-19, -0.9999939076577903929, -0.003490651415223739937 ) ) ;
#6183=ORIENTED_EDGE ( 'NONE', *, *, #93164, .F. ) ;
#6185=CIRCLE ( 'NONE', #8246, 0.06509327318403745899 ) ;
#6186=AXIS2_PLACEMENT_3D ( 'NONE', #8170, #38298, #81278 ) ;
#6187=PLANE ( 'NONE',  #126036 ) ;
#6188=ORIENTED_EDGE ( 'NONE', *, *, #57240, .T. ) ;
#6189=ORIENTED_EDGE ( 'NONE', *, *, #94855, .F. ) ;
#6190=DIRECTION ( 'NONE',  ( 0.000000000000000000, 1.000000000000000000, 0.000000000000000000 ) ) ;
#6191=LINE ( 'NONE', #105708, #5411 ) ;
#6193=FACE_OUTER_BOUND ( 'NONE', #29991, .T. ) ;
#6194=EDGE_CURVE ( 'NONE', #33099, #47526, #6744, .T. ) ;
#6195=DIRECTION ( 'NONE',  ( 0.000000000000000000, 0.000000000000000000, 1.000000000000000000 ) ) ;
#6196=CARTESIAN_POINT ( 'NONE',  ( -1.900000000000034106, 12.50000000000000000, -3.983716857408426293 ) ) ;
#6197=ORIENTED_EDGE ( 'NONE', *, *, #71054, .T. ) ;
#6198=DIRECTION ( 'NONE',  ( 0.000000000000000000, 0.000000000000000000, -1.000000000000000000 ) ) ;
#6199=VECTOR ( 'NONE', #60908, 1000.000000000000000 ) ;
#6200=CONICAL_SURFACE ( 'NONE', #114876, 0.1000000000000002554, 0.003490658503988666988 ) ;
#6201=ORIENTED_EDGE ( 'NONE', *, *, #57822, .F. ) ;
#6202=EDGE_CURVE ( 'NONE', #113352, #36869, #33336, .T. ) ;
#6203=CARTESIAN_POINT ( 'NONE',  ( 6.249999999999934275, 2.500000000000000000, -7.188010851410854052 ) ) ;
#6204=FACE_OUTER_BOUND ( 'NONE', #87816, .T. ) ;
#6205=ADVANCED_FACE ( 'NONE', ( #95804 ), #112745, .T. ) ;
#6206=DIRECTION ( 'NONE',  ( -0.000000000000000000, -1.000000000000000000, -0.000000000000000000 ) ) ;
#6207=CIRCLE ( 'NONE', #91618, 0.06509327318403745899 ) ;
#6208=VERTEX_POINT ( 'NONE', #95166 ) ;
#6209=AXIS2_PLACEMENT_3D ( 'NONE', #65099, #73637, #122116 ) ;
#6210=AXIS2_PLACEMENT_3D ( 'NONE', #120480, #19036, #100819 ) ;
#6211=DIRECTION ( 'NONE',  ( -4.274815082592931898E-19, -0.9999939076577903929, -0.003490651415223739937 ) ) ;
#6212=CARTESIAN_POINT ( 'NONE',  ( -7.700000000000016165, 12.50000000000000000, 0.3464101615137735735 ) ) ;
#6213=ADVANCED_FACE ( 'NONE', ( #114791 ), #41743, .T. ) ;
#6214=AXIS2_PLACEMENT_3D ( 'NONE', #136, #80003, #119934 ) ;
#6215=ORIENTED_EDGE ( 'NONE', *, *, #2136, .T. ) ;
#6216=DIRECTION ( 'NONE',  ( 0.000000000000000000, 0.000000000000000000, 1.000000000000000000 ) ) ;
#6217=CONICAL_SURFACE ( 'NONE', #14625, 0.09999999999999982514, 0.003490658503988666988 ) ;
#6218=ORIENTED_EDGE ( 'NONE', *, *, #117354, .F. ) ;
#6219=VERTEX_POINT ( 'NONE', #34980 ) ;
#6221=VERTEX_POINT ( 'NONE', #54575 ) ;
#6222=CARTESIAN_POINT ( 'NONE',  ( -0.8500000000000390576, 2.500000000000000000, -2.265063509461101798 ) ) ;
#6223=PLANE ( 'NONE',  #12941 ) ;
#6224=DIRECTION ( 'NONE',  ( 0.000000000000000000, 0.000000000000000000, -1.000000000000000000 ) ) ;
#6225=ORIENTED_EDGE ( 'NONE', *, *, #90568, .T. ) ;
#6226=FACE_BOUND ( 'NONE', #106653, .T. ) ;
#6228=EDGE_LOOP ( 'NONE', ( #50551, #78646 ) ) ;
#6229=CIRCLE ( 'NONE', #73066, 0.09999999999999982514 ) ;
#6230=DIRECTION ( 'NONE',  ( 0.000000000000000000, 1.000000000000000000, 0.000000000000000000 ) ) ;
#6231=CARTESIAN_POINT ( 'NONE',  ( -9.600000000000006750, 2.500000000000000000, 5.122947341949749323 ) ) ;
#6232=ORIENTED_EDGE ( 'NONE', *, *, #53840, .F. ) ;
#6233=ADVANCED_FACE ( 'NONE', ( #105634 ), #2001, .T. ) ;
#6234=EDGE_LOOP ( 'NONE', ( #4418, #50719, #44020, #10855 ) ) ;
#6235=ORIENTED_EDGE ( 'NONE', *, *, #96124, .T. ) ;
#6236=DIRECTION ( 'NONE',  ( 0.000000000000000000, 1.000000000000000000, 0.000000000000000000 ) ) ;
#6237=DIRECTION ( 'NONE',  ( 0.000000000000000000, 0.000000000000000000, 1.000000000000000000 ) ) ;
#6238=DIRECTION ( 'NONE',  ( 0.000000000000000000, 0.000000000000000000, 1.000000000000000000 ) ) ;
#6239=ADVANCED_FACE ( 'NONE', ( #65034 ), #114164, .T. ) ;
#6240=FACE_BOUND ( 'NONE', #102700, .T. ) ;
#6241=VERTEX_POINT ( 'NONE', #23857 ) ;
#6243=ADVANCED_FACE ( 'NONE', ( #55247 ), #110670, .T. ) ;
#6244=CARTESIAN_POINT ( 'NONE',  ( -3.150000000000030553, 2.500000000000000000, 6.048780366869520364 ) ) ;
#6245=DIRECTION ( 'NONE',  ( 0.000000000000000000, 1.000000000000000000, 0.000000000000000000 ) ) ;
#6246=DIRECTION ( 'NONE',  ( 0.000000000000000000, 0.000000000000000000, 1.000000000000000000 ) ) ;
#6247=EDGE_CURVE ( 'NONE', #103899, #49433, #26430, .T. ) ;
#6248=CARTESIAN_POINT ( 'NONE',  ( -9.800000000000006040, 2.500000000000000000, 4.576537180435972019 ) ) ;
#6249=ADVANCED_FACE ( 'NONE', ( #25127 ), #18733, .T. ) ;
#6250=FACE_OUTER_BOUND ( 'NONE', #16444, .T. ) ;
#6251=AXIS2_PLACEMENT_3D ( 'NONE', #42080, #45785, #55592 ) ;
#6252=EDGE_CURVE ( 'NONE', #23628, #64551, #6102, .T. ) ;
#6253=DIRECTION ( 'NONE',  ( -0.000000000000000000, -1.000000000000000000, -0.000000000000000000 ) ) ;
#6254=DIRECTION ( 'NONE',  ( -0.000000000000000000, 1.000000000000000000, -0.000000000000000000 ) ) ;
#6255=CARTESIAN_POINT ( 'NONE',  ( -5.000000000000026645, 12.50000000000000000, -3.702399969078687292 ) ) ;
#6256=AXIS2_PLACEMENT_3D ( 'NONE', #33129, #85430, #33753 ) ;
#6257=AXIS2_PLACEMENT_3D ( 'NONE', #63907, #103834, #64541 ) ;
#6258=ADVANCED_FACE ( 'NONE', ( #75509 ), #55874, .T. ) ;
#6259=ORIENTED_EDGE ( 'NONE', *, *, #38213, .F. ) ;
#6260=EDGE_LOOP ( 'NONE', ( #55122, #12281 ) ) ;
#6261=VERTEX_POINT ( 'NONE', #37543 ) ;
#6262=VERTEX_POINT ( 'NONE', #89845 ) ;
#6263=EDGE_LOOP ( 'NONE', ( #87844, #62549 ) ) ;
#6264=CARTESIAN_POINT ( 'NONE',  ( -4.200000000000025935, 2.500000000000000000, 4.230127018922196669 ) ) ;
#6265=CARTESIAN_POINT ( 'NONE',  ( -11.64999999999999680, 2.500000000000000000, 7.188010851410848723 ) ) ;
#6266=ORIENTED_EDGE ( 'NONE', *, *, #38818, .T. ) ;
#6267=FACE_BOUND ( 'NONE', #26959, .T. ) ;
#6268=EDGE_CURVE ( 'NONE', #78915, #39292, #60525, .T. ) ;
#6269=PLANE ( 'NONE',  #33316 ) ;
#6270=CIRCLE ( 'NONE', #94027, 0.06509327318403745899 ) ;
#6271=CARTESIAN_POINT ( 'NONE',  ( 2.099999999999948574, 2.500000000000000000, 4.330127018922196314 ) ) ;
#6272=CARTESIAN_POINT ( 'NONE',  ( -1.450000000000035483, 12.50000000000000000, 6.083687093685483660 ) ) ;
#6273=CARTESIAN_POINT ( 'NONE',  ( -13.34999999999999076, 12.50000000000000000, 2.857883832488652853 ) ) ;
#6274=CARTESIAN_POINT ( 'NONE',  ( 5.849999999999935696, 2.500000000000000000, -6.495190528383302464 ) ) ;
#6277=ORIENTED_EDGE ( 'NONE', *, *, #24596, .F. ) ;
#6278=ORIENTED_EDGE ( 'NONE', *, *, #21936, .T. ) ;
#6279=ORIENTED_EDGE ( 'NONE', *, *, #99567, .F. ) ;
#6280=CARTESIAN_POINT ( 'NONE',  ( 11.44999999999990692, 2.500000000000000000, 1.918653347947321564 ) ) ;
#6281=DIRECTION ( 'NONE',  ( 0.000000000000000000, -0.9999939076577903929, 0.003490651415223739937 ) ) ;
#6282=FACE_OUTER_BOUND ( 'NONE', #2271, .T. ) ;
#6283=ORIENTED_EDGE ( 'NONE', *, *, #90346, .T. ) ;
#6284=CARTESIAN_POINT ( 'NONE',  ( 16.04820284965640909, 1.500000000000000888, -6.585610464672832620 ) ) ;
#6285=VECTOR ( 'NONE', #106630, 1000.000000000000000 ) ;
#6286=DIRECTION ( 'NONE',  ( -4.274815082592931898E-19, -0.9999939076577903929, -0.003490651415223739937 ) ) ;
#6287=AXIS2_PLACEMENT_3D ( 'NONE', #108846, #28377, #19165 ) ;
#6288=DIRECTION ( 'NONE',  ( 0.000000000000000000, 0.000000000000000000, 1.000000000000000000 ) ) ;
#6290=DIRECTION ( 'NONE',  ( 0.000000000000000000, 0.000000000000000000, 1.000000000000000000 ) ) ;
#6291=FACE_OUTER_BOUND ( 'NONE', #39820, .T. ) ;
#6292=ORIENTED_EDGE ( 'NONE', *, *, #106100, .F. ) ;
#6293=CARTESIAN_POINT ( 'NONE',  ( -9.400000000000009237, 12.50000000000000000, -3.918623584224384615 ) ) ;
#6294=CONICAL_SURFACE ( 'NONE', #119196, 0.1000000000000002554, 0.003490658503988666988 ) ;
#6295=ORIENTED_EDGE ( 'NONE', *, *, #30584, .T. ) ;
#6296=ADVANCED_FACE ( 'NONE', ( #36897 ), #16561, .T. ) ;
#6297=ORIENTED_EDGE ( 'NONE', *, *, #15863, .F. ) ;
#6298=FACE_OUTER_BOUND ( 'NONE', #70262, .T. ) ;
#6299=CARTESIAN_POINT ( 'NONE',  ( 10.79999999999991012, 12.50000000000000000, 4.330127018922196314 ) ) ;
#6300=DIRECTION ( 'NONE',  ( 0.000000000000000000, 0.000000000000000000, 1.000000000000000000 ) ) ;
#6301=CONICAL_SURFACE ( 'NONE', #75277, 0.1000000000000002554, 0.003490658503988666988 ) ;
#6302=EDGE_LOOP ( 'NONE', ( #85111, #51502 ) ) ;
#6303=VERTEX_POINT ( 'NONE', #76817 ) ;
#6304=EDGE_CURVE ( 'NONE', #34635, #79439, #116723, .T. ) ;
#6306=DIRECTION ( 'NONE',  ( 0.000000000000000000, 1.000000000000000000, 0.000000000000000000 ) ) ;
#6307=CIRCLE ( 'NONE', #23067, 0.1000000000000002554 ) ;
#6308=LINE ( 'NONE', #17422, #110108 ) ;
#6309=CARTESIAN_POINT ( 'NONE',  ( -10.00000000000000533, 2.500000000000000000, 4.922947341949748257 ) ) ;
#6310=ORIENTED_EDGE ( 'NONE', *, *, #3382, .T. ) ;
#6311=ORIENTED_EDGE ( 'NONE', *, *, #65356, .T. ) ;
#6312=CARTESIAN_POINT ( 'NONE',  ( 7.499999999999925393, 2.500000000000000000, -0.7928203230275542301 ) ) ;
#6313=VERTEX_POINT ( 'NONE', #27071 ) ;
#6314=FACE_OUTER_BOUND ( 'NONE', #114419, .T. ) ;
#6315=CARTESIAN_POINT ( 'NONE',  ( 10.84999999999991260, 12.50000000000000000, 6.495190528383297135 ) ) ;
#6316=EDGE_LOOP ( 'NONE', ( #24358, #31006, #438, #91883 ) ) ;
#6317=DIRECTION ( 'NONE',  ( 0.000000000000000000, 1.000000000000000000, 0.000000000000000000 ) ) ;
#6318=DIRECTION ( 'NONE',  ( -0.000000000000000000, 1.000000000000000000, -0.000000000000000000 ) ) ;
#6319=AXIS2_PLACEMENT_3D ( 'NONE', #26879, #56961, #79216 ) ;
#6320=FACE_OUTER_BOUND ( 'NONE', #87531, .T. ) ;
#6321=LINE ( 'NONE', #106485, #91823 ) ;
#6322=VERTEX_POINT ( 'NONE', #89207 ) ;
#6323=CARTESIAN_POINT ( 'NONE',  ( 7.049999999999930544, 12.50000000000000000, -6.495190528383302464 ) ) ;
#6324=CARTESIAN_POINT ( 'NONE',  ( -8.750000000000010658, 2.500000000000000000, -7.188010851410848723 ) ) ;
#6326=EDGE_LOOP ( 'NONE', ( #40917, #44270, #49656, #83862 ) ) ;
#6328=DIRECTION ( 'NONE',  ( 0.000000000000000000, 1.000000000000000000, 0.000000000000000000 ) ) ;
#6329=CARTESIAN_POINT ( 'NONE',  ( 11.64999999999990798, 12.50000000000000000, -1.537336459617587581 ) ) ;
#6330=CARTESIAN_POINT ( 'NONE',  ( 8.749999999999920064, 2.500000000000000000, 5.802370205355744659 ) ) ;
#6331=DIRECTION ( 'NONE',  ( -0.000000000000000000, -1.000000000000000000, -0.000000000000000000 ) ) ;
#6332=DIRECTION ( 'NONE',  ( -0.000000000000000000, -1.000000000000000000, -0.000000000000000000 ) ) ;
#6333=EDGE_CURVE ( 'NONE', #81732, #87716, #48645, .T. ) ;
#6334=CARTESIAN_POINT ( 'NONE',  ( 0.1999999999999576006, 2.500000000000000000, -4.676537180435978769 ) ) ;
#6335=CARTESIAN_POINT ( 'NONE',  ( 9.349999999999919709, 2.500000000000000000, 2.611473670974873151 ) ) ;
#6336=DIRECTION ( 'NONE',  ( 0.000000000000000000, 0.000000000000000000, -1.000000000000000000 ) ) ;
#6337=VECTOR ( 'NONE', #29222, 1000.000000000000000 ) ;
#6338=AXIS2_PLACEMENT_3D ( 'NONE', #96626, #65893, #76375 ) ;
#6339=CARTESIAN_POINT ( 'NONE',  ( 12.04999999999990479, 2.500000000000000000, 2.065063509461097624 ) ) ;
#6340=EDGE_CURVE ( 'NONE', #31984, #83877, #62577, .T. ) ;
#6341=ORIENTED_EDGE ( 'NONE', *, *, #17805, .F. ) ;
#6342=CIRCLE ( 'NONE', #94114, 0.1000000000000002554 ) ;
#6343=ORIENTED_EDGE ( 'NONE', *, *, #51640, .T. ) ;
#6344=CARTESIAN_POINT ( 'NONE',  ( -4.800000000000024691, 2.500000000000000000, 4.676537180435972552 ) ) ;
#6345=ADVANCED_FACE ( 'NONE', ( #98368 ), #121141, .T. ) ;
#6346=EDGE_LOOP ( 'NONE', ( #784, #76761 ) ) ;
#6347=FACE_OUTER_BOUND ( 'NONE', #86731, .T. ) ;
#6348=ADVANCED_FACE ( 'NONE', ( #119303 ), #10327, .T. ) ;
#6349=DIRECTION ( 'NONE',  ( 0.000000000000000000, 0.000000000000000000, -1.000000000000000000 ) ) ;
#6350=PLANE ( 'NONE',  #110555 ) ;
#6351=VERTEX_POINT ( 'NONE', #17208 ) ;
#6352=CARTESIAN_POINT ( 'NONE',  ( -3.350000000000028955, 2.500000000000000000, -2.065063509461102065 ) ) ;
#6353=EDGE_CURVE ( 'NONE', #89491, #81018, #37529, .T. ) ;
#6354=DIRECTION ( 'NONE',  ( -4.274815082592931898E-19, -0.9999939076577903929, -0.003490651415223739937 ) ) ;
#6355=CARTESIAN_POINT ( 'NONE',  ( -4.400000000000025224, 12.50000000000000000, 3.918623584224382839 ) ) ;
#6356=VERTEX_POINT ( 'NONE', #8689 ) ;
#6357=ADVANCED_FACE ( 'NONE', ( #78109 ), #27054, .T. ) ;
#6358=CARTESIAN_POINT ( 'NONE',  ( -0.8500000000000395017, 12.50000000000000000, 6.560283801567334372 ) ) ;
#6359=VERTEX_POINT ( 'NONE', #118018 ) ;
#6360=EDGE_LOOP ( 'NONE', ( #121206, #127702 ) ) ;
#6361=ORIENTED_EDGE ( 'NONE', *, *, #44553, .T. ) ;
#6362=ORIENTED_EDGE ( 'NONE', *, *, #13925, .T. ) ;
#6363=DIRECTION ( 'NONE',  ( -0.000000000000000000, 1.000000000000000000, -0.000000000000000000 ) ) ;
#6364=FACE_OUTER_BOUND ( 'NONE', #25845, .T. ) ;
#6365=DIRECTION ( 'NONE',  ( 0.000000000000000000, 0.000000000000000000, -1.000000000000000000 ) ) ;
#6366=CARTESIAN_POINT ( 'NONE',  ( -9.400000000000007461, 2.500000000000000000, 3.883716857408420431 ) ) ;
#6367=CIRCLE ( 'NONE', #35655, 0.1000000000000002554 ) ;
#6368=ORIENTED_EDGE ( 'NONE', *, *, #90775, .F. ) ;
#6369=AXIS2_PLACEMENT_3D ( 'NONE', #86834, #67841, #45643 ) ;
#6370=DIRECTION ( 'NONE',  ( 0.000000000000000000, 1.000000000000000000, 0.000000000000000000 ) ) ;
#6371=EDGE_LOOP ( 'NONE', ( #109626, #92049 ) ) ;
#6372=DIRECTION ( 'NONE',  ( 0.000000000000000000, -0.9999939076577903929, 0.003490651415223739937 ) ) ;
#6373=CARTESIAN_POINT ( 'NONE',  ( 9.549999999999915445, 2.500000000000000000, -2.165063509461101710 ) ) ;
#6374=FACE_OUTER_BOUND ( 'NONE', #88000, .T. ) ;
#6375=CARTESIAN_POINT ( 'NONE',  ( 18.78720903128300179, -2.539625591034222918, 4.564429507521819751 ) ) ;
#6376=AXIS2_PLACEMENT_3D ( 'NONE', #23300, #12821, #104449 ) ;
#6377=ORIENTED_EDGE ( 'NONE', *, *, #51164, .T. ) ;
#6378=EDGE_CURVE ( 'NONE', #41663, #104853, #54245, .T. ) ;
#6379=VERTEX_POINT ( 'NONE', #57167 ) ;
#6380=ORIENTED_EDGE ( 'NONE', *, *, #30228, .T. ) ;
#6381=LINE ( 'NONE', #105915, #2204 ) ;
#6382=CARTESIAN_POINT ( 'NONE',  ( 2.099999999999949463, 2.500000000000000000, 0.7928203230275495672 ) ) ;
#6383=DIRECTION ( 'NONE',  ( 0.000000000000000000, 0.000000000000000000, 1.000000000000000000 ) ) ;
#6384=FACE_BOUND ( 'NONE', #126994, .T. ) ;
#6385=CARTESIAN_POINT ( 'NONE',  ( -7.050000000000016698, 12.50000000000000000, -2.230156782645139391 ) ) ;
#6386=DIRECTION ( 'NONE',  ( 0.000000000000000000, 1.000000000000000000, 0.000000000000000000 ) ) ;
#6387=EDGE_CURVE ( 'NONE', #115596, #14399, #24997, .T. ) ;
#6388=DIRECTION ( 'NONE',  ( -4.274815082592931898E-19, -0.9999939076577903929, -0.003490651415223739937 ) ) ;
#6389=CARTESIAN_POINT ( 'NONE',  ( -6.050000000000017586, 12.50000000000000000, 1.818653347947321475 ) ) ;
#6390=CIRCLE ( 'NONE', #29420, 0.1000000000000000472 ) ;
#6391=AXIS2_PLACEMENT_3D ( 'NONE', #23311, #103177, #13490 ) ;
#6392=EDGE_CURVE ( 'NONE', #4409, #71810, #62663, .T. ) ;
#6394=LINE ( 'NONE', #76469, #75912 ) ;
#6395=EDGE_CURVE ( 'NONE', #20773, #90204, #78767, .T. ) ;
#6396=CARTESIAN_POINT ( 'NONE',  ( -2.950000000000029932, 2.500000000000000000, -2.265063509461101798 ) ) ;
#6397=EDGE_CURVE ( 'NONE', #64508, #116018, #29016, .T. ) ;
#6398=CARTESIAN_POINT ( 'NONE',  ( 9.999999999999911182, 12.50000000000000000, 5.022947341949748790 ) ) ;
#6399=EDGE_CURVE ( 'NONE', #33584, #15359, #12468, .T. ) ;
#6400=VERTEX_POINT ( 'NONE', #29646 ) ;
#6401=CONICAL_SURFACE ( 'NONE', #33556, 0.1000000000000002554, 0.003490658503988666988 ) ;
#6402=ORIENTED_EDGE ( 'NONE', *, *, #36594, .T. ) ;
#6403=VERTEX_POINT ( 'NONE', #69559 ) ;
#6404=ORIENTED_EDGE ( 'NONE', *, *, #16180, .F. ) ;
#6405=CARTESIAN_POINT ( 'NONE',  ( -9.150000000000011013, 12.50000000000000000, -5.802370205355744659 ) ) ;
#6406=FACE_BOUND ( 'NONE', #56960, .T. ) ;
#6407=CARTESIAN_POINT ( 'NONE',  ( -14.14999999999998614, 12.50000000000000000, -2.792790559304614284 ) ) ;
#6408=ADVANCED_FACE ( 'NONE', ( #127214 ), #67619, .T. ) ;
#6409=DIRECTION ( 'NONE',  ( -4.274815082592931898E-19, -0.9999939076577903929, -0.003490651415223739937 ) ) ;
#6410=EDGE_CURVE ( 'NONE', #78664, #69133, #29220, .T. ) ;
#6411=ORIENTED_EDGE ( 'NONE', *, *, #9554, .T. ) ;
#6412=DIRECTION ( 'NONE',  ( -0.000000000000000000, 1.000000000000000000, -0.000000000000000000 ) ) ;
#6413=FACE_OUTER_BOUND ( 'NONE', #119717, .T. ) ;
#6414=EDGE_LOOP ( 'NONE', ( #14323, #45218, #67471, #117364 ) ) ;
#6415=CARTESIAN_POINT ( 'NONE',  ( -11.64999999999999680, 12.50000000000000000, 5.802370205355744659 ) ) ;
#6416=CARTESIAN_POINT ( 'NONE',  ( -0.6000000000000388356, 12.50000000000000000, 4.676537180435972552 ) ) ;
#6417=CIRCLE ( 'NONE', #31603, 0.1000000000000002554 ) ;
#6418=VERTEX_POINT ( 'NONE', #20479 ) ;
#6419=CIRCLE ( 'NONE', #115093, 0.1000000000000000472 ) ;
#6420=CARTESIAN_POINT ( 'NONE',  ( 7.099999999999928590, 2.500000000000000000, -4.330127018922201643 ) ) ;
#6421=AXIS2_PLACEMENT_3D ( 'NONE', #117548, #58029, #27912 ) ;
#6422=CARTESIAN_POINT ( 'NONE',  ( 8.549999999999922551, 12.50000000000000000, -6.083687093685488989 ) ) ;
#6423=EDGE_LOOP ( 'NONE', ( #71379, #13587, #44285, #93788 ) ) ;
#6424=CARTESIAN_POINT ( 'NONE',  ( 4.599999999999935696, 12.50000000000000000, 5.022947341949748790 ) ) ;
#6425=CIRCLE ( 'NONE', #48234, 0.06509327318403745899 ) ;
#6426=DIRECTION ( 'NONE',  ( 0.000000000000000000, 0.000000000000000000, -1.000000000000000000 ) ) ;
#6427=EDGE_LOOP ( 'NONE', ( #43668, #291, #88358, #117742 ) ) ;
#6428=CARTESIAN_POINT ( 'NONE',  ( 6.049999999999932321, 2.500000000000000000, 1.718653347947321386 ) ) ;
#6429=ORIENTED_EDGE ( 'NONE', *, *, #10659, .F. ) ;
#6430=AXIS2_PLACEMENT_3D ( 'NONE', #91978, #120155, #61893 ) ;
#6431=ORIENTED_EDGE ( 'NONE', *, *, #38676, .F. ) ;
#6432=DIRECTION ( 'NONE',  ( 0.000000000000000000, 0.000000000000000000, -1.000000000000000000 ) ) ;
#6433=VERTEX_POINT ( 'NONE', #71496 ) ;
#6434=CARTESIAN_POINT ( 'NONE',  ( 5.399999999999934630, 12.50000000000000000, -0.6928203230275542523 ) ) ;
#6435=DIRECTION ( 'NONE',  ( -0.000000000000000000, -1.000000000000000000, -0.000000000000000000 ) ) ;
#6436=ORIENTED_EDGE ( 'NONE', *, *, #94768, .F. ) ;
#6437=ADVANCED_FACE ( 'NONE', ( #102880 ), #68901, .T. ) ;
#6438=CARTESIAN_POINT ( 'NONE',  ( -3.750000000000025757, 2.500000000000000000, -2.957883832488653830 ) ) ;
#6440=FACE_OUTER_BOUND ( 'NONE', #24489, .T. ) ;
#6441=CARTESIAN_POINT ( 'NONE',  ( 12.69999999999989804, 2.500000000000000000, 0.2464101615137735679 ) ) ;
#6442=CARTESIAN_POINT ( 'NONE',  ( 7.299999999999926104, 2.500000000000000000, -3.983716857408426293 ) ) ;
#6443=LINE ( 'NONE', #28063, #129043 ) ;
#6444=ORIENTED_EDGE ( 'NONE', *, *, #126262, .F. ) ;
#6445=EDGE_CURVE ( 'NONE', #5618, #39246, #119088, .T. ) ;
#6446=ORIENTED_EDGE ( 'NONE', *, *, #52449, .F. ) ;
#6447=CONICAL_SURFACE ( 'NONE', #27393, 0.09999999999999982514, 0.003490658503988666988 ) ;
#6448=DIRECTION ( 'NONE',  ( 0.000000000000000000, 0.000000000000000000, 1.000000000000000000 ) ) ;
#6449=CARTESIAN_POINT ( 'NONE',  ( -13.14999999999999147, 2.500000000000000000, 2.511473670974877503 ) ) ;
#6450=DIRECTION ( 'NONE',  ( 0.000000000000000000, 0.000000000000000000, 1.000000000000000000 ) ) ;
#6451=EDGE_LOOP ( 'NONE', ( #127899, #7119, #67171, #70156 ) ) ;
#6452=EDGE_LOOP ( 'NONE', ( #11839, #48250 ) ) ;
#6453=VERTEX_POINT ( 'NONE', #60419 ) ;
#6454=DIRECTION ( 'NONE',  ( -0.000000000000000000, -1.000000000000000000, -0.000000000000000000 ) ) ;
#6455=CONICAL_SURFACE ( 'NONE', #48353, 0.1000000000000002554, 0.003490658503988666988 ) ;
#6456=DIRECTION ( 'NONE',  ( 0.000000000000000000, -0.000000000000000000, 1.000000000000000000 ) ) ;
#6457=AXIS2_PLACEMENT_3D ( 'NONE', #91997, #21990, #61910 ) ;
#6458=CARTESIAN_POINT ( 'NONE',  ( 0.3999999999999628852, 12.50000000000000000, 0.6277270498435143509 ) ) ;
#6460=DIRECTION ( 'NONE',  ( 0.000000000000000000, 0.000000000000000000, -1.000000000000000000 ) ) ;
#6461=DIRECTION ( 'NONE',  ( -4.274815082592931898E-19, -0.9999939076577903929, -0.003490651415223739937 ) ) ;
#6462=LINE ( 'NONE', #97461, #63228 ) ;
#6463=DIRECTION ( 'NONE',  ( -0.000000000000000000, 1.000000000000000000, -0.000000000000000000 ) ) ;
#6464=DIRECTION ( 'NONE',  ( 0.000000000000000000, -0.9999939076577903929, 0.003490651415223739937 ) ) ;
#6465=CARTESIAN_POINT ( 'NONE',  ( 11.89999999999990798, 2.500000000000000000, 4.676537180435972552 ) ) ;
#6466=AXIS2_PLACEMENT_3D ( 'NONE', #102314, #120656, #40171 ) ;
#6467=CIRCLE ( 'NONE', #62937, 0.09999999999999982514 ) ;
#6468=ORIENTED_EDGE ( 'NONE', *, *, #128749, .F. ) ;
#6469=DIRECTION ( 'NONE',  ( 0.000000000000000000, 1.000000000000000000, 0.000000000000000000 ) ) ;
#6470=ORIENTED_EDGE ( 'NONE', *, *, #4044, .T. ) ;
#6471=ORIENTED_EDGE ( 'NONE', *, *, #108780, .F. ) ;
#6472=DIRECTION ( 'NONE',  ( -0.000000000000000000, -1.000000000000000000, -0.000000000000000000 ) ) ;
#6473=DIRECTION ( 'NONE',  ( 0.000000000000000000, 0.000000000000000000, 1.000000000000000000 ) ) ;
#6474=DIRECTION ( 'NONE',  ( -0.000000000000000000, 1.000000000000000000, -0.000000000000000000 ) ) ;
#6475=CONICAL_SURFACE ( 'NONE', #67118, 0.1000000000000002554, 0.003490658503988666988 ) ;
#6476=CARTESIAN_POINT ( 'NONE',  ( -9.550000000000006040, 2.500000000000000000, -2.165063509461101710 ) ) ;
#6477=CIRCLE ( 'NONE', #104786, 0.1000000000000002554 ) ;
#6479=DIRECTION ( 'NONE',  ( 0.000000000000000000, 0.000000000000000000, 1.000000000000000000 ) ) ;
#6480=DIRECTION ( 'NONE',  ( 0.000000000000000000, 0.000000000000000000, 1.000000000000000000 ) ) ;
#6481=DIRECTION ( 'NONE',  ( 0.000000000000000000, -0.9999939076577903929, 0.003490651415223739937 ) ) ;
#6482=VERTEX_POINT ( 'NONE', #32888 ) ;
#6483=CARTESIAN_POINT ( 'NONE',  ( 10.84999999999990905, 12.50000000000000000, -5.867463478539787225 ) ) ;
#6484=AXIS2_PLACEMENT_3D ( 'NONE', #31232, #11568, #10898 ) ;
#6485=DIRECTION ( 'NONE',  ( -0.000000000000000000, 1.000000000000000000, -0.000000000000000000 ) ) ;
#6486=VERTEX_POINT ( 'NONE', #72799 ) ;
#6487=EDGE_CURVE ( 'NONE', #37790, #51184, #26198, .T. ) ;
#6488=ORIENTED_EDGE ( 'NONE', *, *, #982, .F. ) ;
#6489=CIRCLE ( 'NONE', #102664, 0.09999999999999999167 ) ;
#6490=AXIS2_PLACEMENT_3D ( 'NONE', #62707, #63983, #3773 ) ;
#6491=ORIENTED_EDGE ( 'NONE', *, *, #75975, .T. ) ;
#6492=ADVANCED_FACE ( 'NONE', ( #21769 ), #88890, .T. ) ;
#6493=EDGE_LOOP ( 'NONE', ( #105466, #18695, #8857, #57515 ) ) ;
#6494=EDGE_CURVE ( 'NONE', #45172, #96595, #17867, .T. ) ;
#6495=PLANE ( 'NONE',  #123553 ) ;
#6496=DIRECTION ( 'NONE',  ( 0.000000000000000000, 1.000000000000000000, 0.000000000000000000 ) ) ;
#6497=ORIENTED_EDGE ( 'NONE', *, *, #14737, .F. ) ;
#6498=DIRECTION ( 'NONE',  ( -0.000000000000000000, 1.000000000000000000, -0.000000000000000000 ) ) ;
#6499=CARTESIAN_POINT ( 'NONE',  ( 17.50000000000000000, -2.750000000000000444, -3.432456362931489036 ) ) ;
#6500=EDGE_CURVE ( 'NONE', #62269, #62754, #78542, .T. ) ;
#6501=FACE_OUTER_BOUND ( 'NONE', #94225, .T. ) ;
#6502=EDGE_CURVE ( 'NONE', #114203, #1725, #91040, .T. ) ;
#6503=ORIENTED_EDGE ( 'NONE', *, *, #114097, .T. ) ;
#6504=EDGE_CURVE ( 'NONE', #76324, #89801, #22105, .T. ) ;
#6505=CARTESIAN_POINT ( 'NONE',  ( 10.19999999999991225, 12.50000000000000000, -4.676537180435978769 ) ) ;
#6506=PLANE ( 'NONE',  #114691 ) ;
#6507=ORIENTED_EDGE ( 'NONE', *, *, #41884, .F. ) ;
#6508=VERTEX_POINT ( 'NONE', #165 ) ;
#6509=EDGE_LOOP ( 'NONE', ( #47226, #16697 ) ) ;
#6510=CIRCLE ( 'NONE', #23263, 0.06509327318403745899 ) ;
#6512=CIRCLE ( 'NONE', #108935, 0.06509327318403745899 ) ;
#6513=CARTESIAN_POINT ( 'NONE',  ( -5.000000000000022204, 12.50000000000000000, 3.637306695894644726 ) ) ;
#6514=VECTOR ( 'NONE', #22994, 1000.000000000000000 ) ;
#6515=CIRCLE ( 'NONE', #14928, 0.09999999999999982514 ) ;
#6516=AXIS2_PLACEMENT_3D ( 'NONE', #98406, #48047, #29058 ) ;
#6517=ORIENTED_EDGE ( 'NONE', *, *, #62871, .T. ) ;
#6518=DIRECTION ( 'NONE',  ( -0.000000000000000000, -1.000000000000000000, -0.000000000000000000 ) ) ;
#6519=DIRECTION ( 'NONE',  ( 0.000000000000000000, 0.000000000000000000, 1.000000000000000000 ) ) ;
#6520=DIRECTION ( 'NONE',  ( -0.000000000000000000, 1.000000000000000000, -0.000000000000000000 ) ) ;
#6521=PLANE ( 'NONE',  #69180 ) ;
#6522=ORIENTED_EDGE ( 'NONE', *, *, #118697, .F. ) ;
#6523=DIRECTION ( 'NONE',  ( 0.000000000000000000, 1.000000000000000000, 0.000000000000000000 ) ) ;
#6524=ORIENTED_EDGE ( 'NONE', *, *, #117499, .F. ) ;
#6525=ORIENTED_EDGE ( 'NONE', *, *, #127328, .T. ) ;
#6526=ORIENTED_EDGE ( 'NONE', *, *, #72536, .F. ) ;
#6527=DIRECTION ( 'NONE',  ( 0.000000000000000000, 0.000000000000000000, -1.000000000000000000 ) ) ;
#6528=FACE_BOUND ( 'NONE', #8316, .T. ) ;
#6529=CARTESIAN_POINT ( 'NONE',  ( -10.80000000000000071, 2.500000000000000000, -0.1000000000000022815 ) ) ;
#6530=DIRECTION ( 'NONE',  ( 0.000000000000000000, 1.000000000000000000, 0.000000000000000000 ) ) ;
#6531=DIRECTION ( 'NONE',  ( 0.000000000000000000, 0.000000000000000000, -1.000000000000000000 ) ) ;
#6532=ADVANCED_FACE ( 'NONE', ( #11928 ), #36678, .T. ) ;
#6533=VERTEX_POINT ( 'NONE', #62340 ) ;
#6534=EDGE_CURVE ( 'NONE', #118617, #125586, #28351, .T. ) ;
#6535=CARTESIAN_POINT ( 'NONE',  ( 3.149999999999946176, 12.50000000000000000, -1.818653347947325916 ) ) ;
#6536=DIRECTION ( 'NONE',  ( 0.000000000000000000, 1.000000000000000000, 0.000000000000000000 ) ) ;
#6537=CARTESIAN_POINT ( 'NONE',  ( -0.6500000000000403233, 2.500000000000000000, 1.918653347947321564 ) ) ;
#6538=ADVANCED_FACE ( 'NONE', ( #70220 ), #57600, .T. ) ;
#6539=DIRECTION ( 'NONE',  ( 0.000000000000000000, -0.9999939076577903929, 0.003490651415223739937 ) ) ;
#6540=ORIENTED_EDGE ( 'NONE', *, *, #115589, .F. ) ;
#6541=AXIS2_PLACEMENT_3D ( 'NONE', #27957, #8300, #7655 ) ;
#6542=CARTESIAN_POINT ( 'NONE',  ( 5.649999999999934630, 2.500000000000000000, 6.941600689897073018 ) ) ;
#6543=AXIS2_PLACEMENT_3D ( 'NONE', #95226, #114839, #97793 ) ;
#6545=EDGE_CURVE ( 'NONE', #98108, #100426, #41420, .T. ) ;
#6546=EDGE_LOOP ( 'NONE', ( #3089, #30733 ) ) ;
#6547=LINE ( 'NONE', #83232, #56511 ) ;
#6548=EDGE_CURVE ( 'NONE', #69648, #7472, #55442, .T. ) ;
#6549=DIRECTION ( 'NONE',  ( -0.000000000000000000, -1.000000000000000000, -0.000000000000000000 ) ) ;
#6550=FACE_BOUND ( 'NONE', #82283, .T. ) ;
#6551=AXIS2_PLACEMENT_3D ( 'NONE', #85116, #15724, #35386 ) ;
#6552=FACE_OUTER_BOUND ( 'NONE', #95018, .T. ) ;
#6553=EDGE_CURVE ( 'NONE', #65577, #10375, #105621, .T. ) ;
#6554=AXIS2_PLACEMENT_3D ( 'NONE', #15673, #65430, #45168 ) ;
#6555=EDGE_CURVE ( 'NONE', #109761, #117860, #126550, .T. ) ;
#6556=EDGE_CURVE ( 'NONE', #116101, #78026, #45082, .T. ) ;
#6557=ORIENTED_EDGE ( 'NONE', *, *, #40144, .T. ) ;
#6558=CIRCLE ( 'NONE', #115330, 0.06509327318403745899 ) ;
#6559=CARTESIAN_POINT ( 'NONE',  ( -3.150000000000030109, 2.500000000000000000, -2.511473670974877948 ) ) ;
#6560=DIRECTION ( 'NONE',  ( -0.000000000000000000, -1.000000000000000000, -0.000000000000000000 ) ) ;
#6561=ORIENTED_EDGE ( 'NONE', *, *, #89308, .T. ) ;
#6562=( BOUNDED_CURVE ( )  B_SPLINE_CURVE ( 2, ( #18099, #59347, #10225 ),
 .UNSPECIFIED., .F., .F. ) 
 B_SPLINE_CURVE_WITH_KNOTS ( ( 3, 3 ),
 ( 0.000000000000000000, 8.005299705368666859E-05 ),
 .UNSPECIFIED. ) 
 CURVE ( )  GEOMETRIC_REPRESENTATION_ITEM ( )  RATIONAL_B_SPLINE_CURVE ( ( 1.000000000000000000, 0.9972072019273802157, 0.9944676636817105786 ) ) 
 REPRESENTATION_ITEM ( '' )  );
#6565=ADVANCED_FACE ( 'NONE', ( #122544 ), #82647, .T. ) ;
#6566=ORIENTED_EDGE ( 'NONE', *, *, #51665, .T. ) ;
#6568=CARTESIAN_POINT ( 'NONE',  ( 12.69999999999989804, 2.500000000000000000, 0.3464101615137735735 ) ) ;
#6570=AXIS2_PLACEMENT_3D ( 'NONE', #17853, #27660, #77425 ) ;
#6571=CIRCLE ( 'NONE', #29593, 0.06509327318403745899 ) ;
#6573=CARTESIAN_POINT ( 'NONE',  ( 10.84999999999991260, 2.500000000000000000, -2.757883832488654097 ) ) ;
#6575=ORIENTED_EDGE ( 'NONE', *, *, #22355, .F. ) ;
#6576=DIRECTION ( 'NONE',  ( 0.000000000000000000, 1.000000000000000000, 0.000000000000000000 ) ) ;
#6577=CIRCLE ( 'NONE', #79781, 0.09999999999999982514 ) ;
#6578=FACE_OUTER_BOUND ( 'NONE', #43131, .T. ) ;
#6579=CARTESIAN_POINT ( 'NONE',  ( -9.800000000000006040, 2.500000000000000000, -4.776537180435973973 ) ) ;
#6580=CARTESIAN_POINT ( 'NONE',  ( -1.650000000000034772, 2.500000000000000000, 1.472243186433545459 ) ) ;
#6581=ORIENTED_EDGE ( 'NONE', *, *, #66384, .T. ) ;
#6582=ORIENTED_EDGE ( 'NONE', *, *, #109428, .F. ) ;
#6583=FACE_BOUND ( 'NONE', #9146, .T. ) ;
#6584=EDGE_LOOP ( 'NONE', ( #52544, #19070, #105238, #83919 ) ) ;
#6585=DIRECTION ( 'NONE',  ( -0.000000000000000000, 1.000000000000000000, -0.000000000000000000 ) ) ;
#6586=DIRECTION ( 'NONE',  ( 0.000000000000000000, -0.9999939076577903929, 0.003490651415223739937 ) ) ;
#6587=EDGE_LOOP ( 'NONE', ( #99362, #25948 ) ) ;
#6588=CARTESIAN_POINT ( 'NONE',  ( -10.40000000000000213, 2.500000000000000000, 0.5928203230275495006 ) ) ;
#6589=CARTESIAN_POINT ( 'NONE',  ( 0.8499999999999553468, 12.50000000000000000, 2.165063509461097713 ) ) ;
#6590=DIRECTION ( 'NONE',  ( 0.000000000000000000, 0.000000000000000000, 1.000000000000000000 ) ) ;
#6591=FACE_OUTER_BOUND ( 'NONE', #55548, .T. ) ;
#6592=ORIENTED_EDGE ( 'NONE', *, *, #106322, .F. ) ;
#6593=DIRECTION ( 'NONE',  ( -0.000000000000000000, 1.000000000000000000, -0.000000000000000000 ) ) ;
#6594=DIRECTION ( 'NONE',  ( -0.000000000000000000, -1.000000000000000000, -0.000000000000000000 ) ) ;
#6596=DIRECTION ( 'NONE',  ( 0.000000000000000000, 0.000000000000000000, 1.000000000000000000 ) ) ;
#6597=DIRECTION ( 'NONE',  ( 0.000000000000000000, 1.000000000000000000, 0.000000000000000000 ) ) ;
#6598=VERTEX_POINT ( 'NONE', #26276 ) ;
#6599=EDGE_CURVE ( 'NONE', #105502, #56688, #109820, .T. ) ;
#6600=ORIENTED_EDGE ( 'NONE', *, *, #25923, .T. ) ;
#6601=CARTESIAN_POINT ( 'NONE',  ( -5.850000000000021849, 12.50000000000000000, -1.407149913249512663 ) ) ;
#6602=ORIENTED_EDGE ( 'NONE', *, *, #4953, .F. ) ;
#6603=AXIS2_PLACEMENT_3D ( 'NONE', #1751, #20762, #111719 ) ;
#6604=DIRECTION ( 'NONE',  ( -0.000000000000000000, -1.000000000000000000, -0.000000000000000000 ) ) ;
#6605=CONICAL_SURFACE ( 'NONE', #10819, 0.1000000000000002554, 0.003490658503988666988 ) ;
#6606=CIRCLE ( 'NONE', #98560, 0.1000000000000002554 ) ;
#6607=ORIENTED_EDGE ( 'NONE', *, *, #2981, .F. ) ;
#6608=EDGE_LOOP ( 'NONE', ( #50453, #66755, #8810, #1426 ) ) ;
#6609=ORIENTED_EDGE ( 'NONE', *, *, #77091, .F. ) ;
#6610=DIRECTION ( 'NONE',  ( 0.000000000000000000, 1.000000000000000000, 0.000000000000000000 ) ) ;
#6611=DIRECTION ( 'NONE',  ( 0.000000000000000000, 1.000000000000000000, 0.000000000000000000 ) ) ;
#6612=VECTOR ( 'NONE', #82419, 1000.000000000000000 ) ;
#6613=DIRECTION ( 'NONE',  ( 0.000000000000000000, 0.000000000000000000, 1.000000000000000000 ) ) ;
#6614=AXIS2_PLACEMENT_3D ( 'NONE', #47880, #37415, #74272 ) ;
#6615=CARTESIAN_POINT ( 'NONE',  ( 1.449999999999952216, 12.50000000000000000, -2.511473670974877948 ) ) ;
#6616=CARTESIAN_POINT ( 'NONE',  ( -7.050000000000016698, 2.500000000000000000, -2.165063509461101710 ) ) ;
#6617=CIRCLE ( 'NONE', #33840, 0.06509327318403745899 ) ;
#6618=DIRECTION ( 'NONE',  ( 0.000000000000000000, 1.000000000000000000, 0.000000000000000000 ) ) ;
#6619=VERTEX_POINT ( 'NONE', #123191 ) ;
#6620=DIRECTION ( 'NONE',  ( 0.000000000000000000, 0.000000000000000000, 1.000000000000000000 ) ) ;
#6623=ORIENTED_EDGE ( 'NONE', *, *, #14945, .T. ) ;
#6624=EDGE_LOOP ( 'NONE', ( #45357, #1540 ) ) ;
#6625=ORIENTED_EDGE ( 'NONE', *, *, #38352, .T. ) ;
#6626=DIRECTION ( 'NONE',  ( 0.000000000000000000, 0.000000000000000000, 1.000000000000000000 ) ) ;
#6627=ORIENTED_EDGE ( 'NONE', *, *, #94490, .T. ) ;
#6628=VERTEX_POINT ( 'NONE', #75354 ) ;
#6629=DIRECTION ( 'NONE',  ( 0.000000000000000000, 1.000000000000000000, 0.000000000000000000 ) ) ;
#6630=CARTESIAN_POINT ( 'NONE',  ( 12.29999999999990301, 2.500000000000000000, -0.4464101615137782142 ) ) ;
#6631=CARTESIAN_POINT ( 'NONE',  ( -5.650000000000019895, 12.50000000000000000, 1.818653347947321475 ) ) ;
#6632=DIRECTION ( 'NONE',  ( 0.000000000000000000, 1.000000000000000000, 0.000000000000000000 ) ) ;
#6633=DIRECTION ( 'NONE',  ( -0.000000000000000000, -1.000000000000000000, -0.000000000000000000 ) ) ;
#6634=ORIENTED_EDGE ( 'NONE', *, *, #8310, .F. ) ;
#6635=DIRECTION ( 'NONE',  ( 0.000000000000000000, 0.000000000000000000, 1.000000000000000000 ) ) ;
#6636=AXIS2_PLACEMENT_3D ( 'NONE', #74967, #52741, #122154 ) ;
#6637=CONICAL_SURFACE ( 'NONE', #54679, 0.09999999999999999167, 0.003490658503988666988 ) ;
#6638=VERTEX_POINT ( 'NONE', #113354 ) ;
#6639=DIRECTION ( 'NONE',  ( 0.000000000000000000, 0.000000000000000000, 1.000000000000000000 ) ) ;
#6640=ADVANCED_FACE ( 'NONE', ( #14492 ), #65897, .T. ) ;
#6641=EDGE_LOOP ( 'NONE', ( #74783, #94757 ) ) ;
#6642=DIRECTION ( 'NONE',  ( 0.000000000000000000, 0.000000000000000000, -1.000000000000000000 ) ) ;
#6643=ORIENTED_EDGE ( 'NONE', *, *, #21784, .T. ) ;
#6644=ADVANCED_FACE ( 'NONE', ( #114637 ), #95652, .T. ) ;
#6645=ORIENTED_EDGE ( 'NONE', *, *, #51280, .F. ) ;
#6646=AXIS2_PLACEMENT_3D ( 'NONE', #2358, #32519, #23303 ) ;
#6647=ADVANCED_FACE ( 'NONE', ( #64888 ), #128628, .T. ) ;
#6648=DIRECTION ( 'NONE',  ( 0.000000000000000000, 1.000000000000000000, 0.000000000000000000 ) ) ;
#6649=PLANE ( 'NONE',  #119547 ) ;
#6650=AXIS2_PLACEMENT_3D ( 'NONE', #52699, #122098, #70413 ) ;
#6651=AXIS2_PLACEMENT_3D ( 'NONE', #37455, #45987, #56427 ) ;
#6652=LINE ( 'NONE', #126475, #13170 ) ;
#6653=CARTESIAN_POINT ( 'NONE',  ( 0.1999999999999567124, 2.500000000000000000, -4.083716857408426826 ) ) ;
#6654=ADVANCED_FACE ( 'NONE', ( #23692 ), #93112, .T. ) ;
#6655=CARTESIAN_POINT ( 'NONE',  ( 13.74999999999993427, 2.500000000000000000, 2.165063509461097713 ) ) ;
#6656=EDGE_CURVE ( 'NONE', #36089, #120893, #122353, .T. ) ;
#6657=EDGE_LOOP ( 'NONE', ( #46361, #6592 ) ) ;
#6658=CARTESIAN_POINT ( 'NONE',  ( -7.500000000000013323, 12.50000000000000000, 5.022947341949748790 ) ) ;
#6659=DIRECTION ( 'NONE',  ( 0.000000000000000000, 0.000000000000000000, 1.000000000000000000 ) ) ;
#6660=ADVANCED_FACE ( 'NONE', ( #44621 ), #95153, .T. ) ;
#6661=CARTESIAN_POINT ( 'NONE',  ( -3.300000000000027800, 2.500000000000000000, -4.330127018922201643 ) ) ;
#6662=ADVANCED_FACE ( 'NONE', ( #45919 ), #73424, .T. ) ;
#6663=ADVANCED_FACE ( 'NONE', ( #5328 ), #116072, .T. ) ;
#6664=CARTESIAN_POINT ( 'NONE',  ( -0.4500000000000402012, 12.50000000000000000, 2.165063509461097713 ) ) ;
#6665=CIRCLE ( 'NONE', #40162, 0.1000000000000002554 ) ;
#6666=AXIS2_PLACEMENT_3D ( 'NONE', #51203, #89819, #91115 ) ;
#6667=CARTESIAN_POINT ( 'NONE',  ( -6.900000000000019007, 2.500000000000000000, -4.676537180435978769 ) ) ;
#6668=VERTEX_POINT ( 'NONE', #34165 ) ;
#6669=AXIS2_PLACEMENT_3D ( 'NONE', #115390, #36875, #114769 ) ;
#6670=VECTOR ( 'NONE', #83591, 1000.000000000000000 ) ;
#6671=EDGE_LOOP ( 'NONE', ( #57556, #104047, #95892, #93036 ) ) ;
#6672=CARTESIAN_POINT ( 'NONE',  ( -9.999999999999971578, 2.500000000000000000, -4.230127018922197557 ) ) ;
#6673=EDGE_CURVE ( 'NONE', #58516, #125196, #3220, .T. ) ;
#6674=AXIS2_PLACEMENT_3D ( 'NONE', #73547, #54547, #46506 ) ;
#6675=ORIENTED_EDGE ( 'NONE', *, *, #110974, .T. ) ;
#6676=DIRECTION ( 'NONE',  ( -0.000000000000000000, -1.000000000000000000, -0.000000000000000000 ) ) ;
#6677=DIRECTION ( 'NONE',  ( 0.000000000000000000, 1.000000000000000000, 0.000000000000000000 ) ) ;
#6679=ORIENTED_EDGE ( 'NONE', *, *, #126610, .T. ) ;
#6681=DIRECTION ( 'NONE',  ( 0.000000000000000000, 0.000000000000000000, 1.000000000000000000 ) ) ;
#6682=CARTESIAN_POINT ( 'NONE',  ( -6.050000000000017586, 12.50000000000000000, 6.213873640053558134 ) ) ;
#6683=DIRECTION ( 'NONE',  ( 0.000000000000000000, 1.000000000000000000, 0.000000000000000000 ) ) ;
#6684=EDGE_LOOP ( 'NONE', ( #99168, #115384, #53763, #93789 ) ) ;
#6685=DIRECTION ( 'NONE',  ( 0.000000000000000000, 1.000000000000000000, 0.000000000000000000 ) ) ;
#6686=DIRECTION ( 'NONE',  ( 0.000000000000000000, 1.000000000000000000, 0.000000000000000000 ) ) ;
#6687=ORIENTED_EDGE ( 'NONE', *, *, #75700, .F. ) ;
#6688=CARTESIAN_POINT ( 'NONE',  ( 11.04999999999991189, 12.50000000000000000, 6.148780366869520897 ) ) ;
#6689=CARTESIAN_POINT ( 'NONE',  ( 0.8499999999999545697, 2.500000000000000000, -1.572243186433550211 ) ) ;
#6690=CARTESIAN_POINT ( 'NONE',  ( -3.550000000000028244, 12.50000000000000000, 2.576566944158910744 ) ) ;
#6691=EDGE_LOOP ( 'NONE', ( #9714, #3701, #40850, #99585 ) ) ;
#6692=DIRECTION ( 'NONE',  ( 0.000000000000000000, 0.000000000000000000, 1.000000000000000000 ) ) ;
#6693=CONICAL_SURFACE ( 'NONE', #73621, 0.09999999999999999167, 0.003490658503988666988 ) ;
#6694=CIRCLE ( 'NONE', #79895, 0.06509327318403743123 ) ;
#6695=CIRCLE ( 'NONE', #111176, 0.06509327318403745899 ) ;
#6696=VERTEX_POINT ( 'NONE', #114013 ) ;
#6697=ADVANCED_FACE ( 'NONE', ( #45272 ), #24339, .T. ) ;
#6698=CARTESIAN_POINT ( 'NONE',  ( -11.64999999999999680, 2.500000000000000000, -7.288010851410851032 ) ) ;
#6699=DIRECTION ( 'NONE',  ( 0.000000000000000000, 0.000000000000000000, -1.000000000000000000 ) ) ;
#6700=DIRECTION ( 'NONE',  ( 0.000000000000000000, 0.000000000000000000, 1.000000000000000000 ) ) ;
#6701=EDGE_CURVE ( 'NONE', #72606, #76567, #70121, .T. ) ;
#6702=VERTEX_POINT ( 'NONE', #84543 ) ;
#6703=VECTOR ( 'NONE', #112834, 1000.000000000000000 ) ;
#6704=LINE ( 'NONE', #86583, #55195 ) ;
#6705=CONICAL_SURFACE ( 'NONE', #2517, 0.1000000000000000472, 0.003490658503988666988 ) ;
#6706=EDGE_CURVE ( 'NONE', #69018, #40490, #124474, .T. ) ;
#6707=AXIS2_PLACEMENT_3D ( 'NONE', #31458, #93591, #92291 ) ;
#6708=AXIS2_PLACEMENT_3D ( 'NONE', #87914, #89228, #8080 ) ;
#6709=ORIENTED_EDGE ( 'NONE', *, *, #56234, .F. ) ;
#6710=AXIS2_PLACEMENT_3D ( 'NONE', #70573, #39852, #89568 ) ;
#6711=EDGE_CURVE ( 'NONE', #43890, #93582, #55085, .T. ) ;
#6712=ORIENTED_EDGE ( 'NONE', *, *, #44526, .F. ) ;
#6713=CIRCLE ( 'NONE', #84107, 0.06509327318403745899 ) ;
#6714=CARTESIAN_POINT ( 'NONE',  ( 7.499999999999925393, 2.500000000000000000, 4.922947341949748257 ) ) ;
#6715=EDGE_CURVE ( 'NONE', #2794, #86533, #105715, .T. ) ;
#6716=EDGE_CURVE ( 'NONE', #119339, #5078, #32573, .T. ) ;
#6717=EDGE_LOOP ( 'NONE', ( #89397, #39942 ) ) ;
#6718=DIRECTION ( 'NONE',  ( 0.000000000000000000, 0.000000000000000000, 1.000000000000000000 ) ) ;
#6719=DIRECTION ( 'NONE',  ( 0.000000000000000000, 0.000000000000000000, 1.000000000000000000 ) ) ;
#6720=ORIENTED_EDGE ( 'NONE', *, *, #43202, .T. ) ;
#6721=EDGE_LOOP ( 'NONE', ( #80549, #97148, #114257, #33417 ) ) ;
#6722=CARTESIAN_POINT ( 'NONE',  ( -8.150000000000014566, 2.500000000000000000, -6.248780366869521430 ) ) ;
#6723=DIRECTION ( 'NONE',  ( 0.000000000000000000, 1.000000000000000000, 0.000000000000000000 ) ) ;
#6724=EDGE_LOOP ( 'NONE', ( #99634, #100338 ) ) ;
#6725=ADVANCED_FACE ( 'NONE', ( #56361 ), #108041, .T. ) ;
#6726=FACE_OUTER_BOUND ( 'NONE', #110354, .T. ) ;
#6727=DIRECTION ( 'NONE',  ( -4.274815082592931898E-19, -0.9999939076577903929, -0.003490651415223739937 ) ) ;
#6728=CARTESIAN_POINT ( 'NONE',  ( 17.45652781226495875, -2.453230724138371954, -4.494708854621484839 ) ) ;
#6729=LINE ( 'NONE', #35594, #113569 ) ;
#6730=DIRECTION ( 'NONE',  ( 0.000000000000000000, -0.9999939076577903929, 0.003490651415223739937 ) ) ;
#6731=DIRECTION ( 'NONE',  ( 0.000000000000000000, 0.000000000000000000, 1.000000000000000000 ) ) ;
#6732=CIRCLE ( 'NONE', #23491, 0.09999999999999982514 ) ;
#6733=ORIENTED_EDGE ( 'NONE', *, *, #60576, .F. ) ;
#6734=EDGE_LOOP ( 'NONE', ( #14271, #52690, #121581, #9561 ) ) ;
#6735=VERTEX_POINT ( 'NONE', #76658 ) ;
#6736=ORIENTED_EDGE ( 'NONE', *, *, #112977, .F. ) ;
#6737=CARTESIAN_POINT ( 'NONE',  ( -13.94999999999998863, 12.50000000000000000, 2.511473670974877503 ) ) ;
#6738=CARTESIAN_POINT ( 'NONE',  ( -11.24999999999996447, 2.500000000000000000, -6.395190528383298378 ) ) ;
#6739=DIRECTION ( 'NONE',  ( 0.000000000000000000, 0.000000000000000000, 1.000000000000000000 ) ) ;
#6740=ORIENTED_EDGE ( 'NONE', *, *, #32620, .F. ) ;
#6741=FACE_BOUND ( 'NONE', #29353, .T. ) ;
#6742=EDGE_CURVE ( 'NONE', #118052, #83264, #126644, .T. ) ;
#6743=AXIS2_PLACEMENT_3D ( 'NONE', #28481, #89332, #97847 ) ;
#6744=LINE ( 'NONE', #104338, #91897 ) ;
#6745=DIRECTION ( 'NONE',  ( 0.000000000000000000, 1.000000000000000000, 0.000000000000000000 ) ) ;
#6746=AXIS2_PLACEMENT_3D ( 'NONE', #86667, #47406, #28409 ) ;
#6747=AXIS2_PLACEMENT_3D ( 'NONE', #1468, #9367, #99693 ) ;
#6748=CARTESIAN_POINT ( 'NONE',  ( 2.099999999999948574, 2.500000000000000000, 3.637306695894644726 ) ) ;
#6749=AXIS2_PLACEMENT_3D ( 'NONE', #120049, #111504, #80120 ) ;
#6750=CARTESIAN_POINT ( 'NONE',  ( -7.300000000000016698, 2.500000000000000000, -4.676537180435978769 ) ) ;
#6751=CARTESIAN_POINT ( 'NONE',  ( 10.59999999999990905, 12.50000000000000000, 4.741630453620009789 ) ) ;
#6752=PLANE ( 'NONE',  #104022 ) ;
#6753=DIRECTION ( 'NONE',  ( 0.000000000000000000, 1.000000000000000000, 0.000000000000000000 ) ) ;
#6754=FACE_OUTER_BOUND ( 'NONE', #26727, .T. ) ;
#6755=CARTESIAN_POINT ( 'NONE',  ( -0.4000000000000331624, 12.50000000000000000, 0.000000000000000000 ) ) ;
#6756=CIRCLE ( 'NONE', #107029, 0.06509327318403745899 ) ;
#6757=LINE ( 'NONE', #93895, #20893 ) ;
#6758=AXIS2_PLACEMENT_3D ( 'NONE', #20441, #80002, #30280 ) ;
#6759=VERTEX_POINT ( 'NONE', #38018 ) ;
#6761=EDGE_CURVE ( 'NONE', #83109, #935, #59762, .T. ) ;
#6762=VERTEX_POINT ( 'NONE', #87110 ) ;
#6763=CONICAL_SURFACE ( 'NONE', #52757, 0.09999999999999982514, 0.003490658503988666988 ) ;
#6764=VERTEX_POINT ( 'NONE', #116567 ) ;
#6765=AXIS2_PLACEMENT_3D ( 'NONE', #70104, #41941, #79918 ) ;
#6766=AXIS2_PLACEMENT_3D ( 'NONE', #77311, #48497, #7914 ) ;
#6767=CARTESIAN_POINT ( 'NONE',  ( 3.949999999999941558, 12.50000000000000000, -6.148780366869526226 ) ) ;
#6768=DIRECTION ( 'NONE',  ( -4.274815082592931898E-19, -0.9999939076577903929, -0.003490651415223739937 ) ) ;
#6769=ORIENTED_EDGE ( 'NONE', *, *, #44076, .F. ) ;
#6770=VERTEX_POINT ( 'NONE', #8534 ) ;
#6771=ORIENTED_EDGE ( 'NONE', *, *, #95816, .T. ) ;
#6772=CIRCLE ( 'NONE', #123863, 0.06509327318403745899 ) ;
#6773=CARTESIAN_POINT ( 'NONE',  ( 0.4499999999999552136, 2.500000000000000000, 6.395190528383296602 ) ) ;
#6774=CIRCLE ( 'NONE', #86205, 0.1000000000000002554 ) ;
#6775=CARTESIAN_POINT ( 'NONE',  ( 8.512291507278442637, -1.500000000000000222, 9.502944100741331113 ) ) ;
#6776=DIRECTION ( 'NONE',  ( 0.000000000000000000, 0.000000000000000000, 1.000000000000000000 ) ) ;
#6777=CARTESIAN_POINT ( 'NONE',  ( -3.100000000000028511, 12.50000000000000000, 0.2813168883297362810 ) ) ;
#6779=EDGE_CURVE ( 'NONE', #108500, #69856, #36771, .T. ) ;
#6780=ORIENTED_EDGE ( 'NONE', *, *, #36732, .T. ) ;
#6781=EDGE_LOOP ( 'NONE', ( #5148, #9228, #101139, #91964 ) ) ;
#6782=ORIENTED_EDGE ( 'NONE', *, *, #29320, .F. ) ;
#6783=ORIENTED_EDGE ( 'NONE', *, *, #11565, .T. ) ;
#6785=AXIS2_PLACEMENT_3D ( 'NONE', #22965, #49860, #101523 ) ;
#6786=ORIENTED_EDGE ( 'NONE', *, *, #30374, .T. ) ;
#6787=ORIENTED_EDGE ( 'NONE', *, *, #56026, .F. ) ;
#6788=FACE_OUTER_BOUND ( 'NONE', #83110, .T. ) ;
#6789=FACE_OUTER_BOUND ( 'NONE', #78288, .T. ) ;
#6790=DIRECTION ( 'NONE',  ( 0.000000000000000000, 0.000000000000000000, 1.000000000000000000 ) ) ;
#6791=AXIS2_PLACEMENT_3D ( 'NONE', #18017, #45568, #105768 ) ;
#6792=FACE_OUTER_BOUND ( 'NONE', #103509, .T. ) ;
#6794=AXIS2_PLACEMENT_3D ( 'NONE', #45812, #85714, #6479 ) ;
#6795=DIRECTION ( 'NONE',  ( 0.000000000000000000, 1.000000000000000000, 0.000000000000000000 ) ) ;
#6796=ORIENTED_EDGE ( 'NONE', *, *, #23589, .F. ) ;
#6797=LINE ( 'NONE', #15341, #90817 ) ;
#6798=AXIS2_PLACEMENT_3D ( 'NONE', #1354, #22946, #12462 ) ;
#6799=AXIS2_PLACEMENT_3D ( 'NONE', #13613, #53559, #3807 ) ;
#6800=EDGE_LOOP ( 'NONE', ( #110603, #78866, #89663, #95867 ) ) ;
#6802=AXIS2_PLACEMENT_3D ( 'NONE', #33122, #84121, #124053 ) ;
#6803=EDGE_CURVE ( 'NONE', #6219, #66296, #53487, .T. ) ;
#6804=ORIENTED_EDGE ( 'NONE', *, *, #8550, .T. ) ;
#6805=CARTESIAN_POINT ( 'NONE',  ( 9.349999999999916156, 12.50000000000000000, -1.818653347947326138 ) ) ;
#6806=LINE ( 'NONE', #86686, #42820 ) ;
#6807=CONICAL_SURFACE ( 'NONE', #94654, 0.09999999999999982514, 0.003490658503988666988 ) ;
#6808=EDGE_LOOP ( 'NONE', ( #333, #42894 ) ) ;
#6809=AXIS2_PLACEMENT_3D ( 'NONE', #62059, #121594, #82988 ) ;
#6810=CARTESIAN_POINT ( 'NONE',  ( 3.549999999999944755, 12.50000000000000000, -2.511473670974877948 ) ) ;
#6811=LINE ( 'NONE', #77514, #12185 ) ;
#6812=EDGE_LOOP ( 'NONE', ( #16203, #103969, #101660, #63309 ) ) ;
#6813=ADVANCED_FACE ( 'NONE', ( #118503 ), #70203, .T. ) ;
#6814=DIRECTION ( 'NONE',  ( -0.000000000000000000, 1.000000000000000000, -0.000000000000000000 ) ) ;
#6816=EDGE_CURVE ( 'NONE', #100735, #2439, #68760, .T. ) ;
#6817=ADVANCED_FACE ( 'NONE', ( #77939 ), #39893, .T. ) ;
#6818=ORIENTED_EDGE ( 'NONE', *, *, #76349, .T. ) ;
#6819=CARTESIAN_POINT ( 'NONE',  ( -6.249999999999984901, 12.50000000000000000, -2.165063509461101710 ) ) ;
#6820=CARTESIAN_POINT ( 'NONE',  ( 6.249999999999930722, 12.50000000000000000, 1.537336459617582918 ) ) ;
#6821=EDGE_CURVE ( 'NONE', #73823, #69623, #40982, .T. ) ;
#6823=ADVANCED_FACE ( 'NONE', ( #17047 ), #56998, .T. ) ;
#6825=DIRECTION ( 'NONE',  ( 0.000000000000000000, 0.000000000000000000, 1.000000000000000000 ) ) ;
#6826=ADVANCED_FACE ( 'NONE', ( #127055 ), #72271, .T. ) ;
#6827=FACE_OUTER_BOUND ( 'NONE', #43561, .T. ) ;
#6828=EDGE_CURVE ( 'NONE', #79421, #11460, #57692, .T. ) ;
#6829=EDGE_CURVE ( 'NONE', #37333, #92919, #114110, .T. ) ;
#6830=CIRCLE ( 'NONE', #80021, 0.1000000000000002554 ) ;
#6831=EDGE_LOOP ( 'NONE', ( #4269, #57537, #50905, #35957 ) ) ;
#6832=ADVANCED_FACE ( 'NONE', ( #71328 ), #111243, .T. ) ;
#6833=CARTESIAN_POINT ( 'NONE',  ( 11.69999999999990514, 12.50000000000000000, 0.06509327318403515528 ) ) ;
#6834=EDGE_CURVE ( 'NONE', #56267, #118565, #20039, .T. ) ;
#6835=VERTEX_POINT ( 'NONE', #21605 ) ;
#6836=CARTESIAN_POINT ( 'NONE',  ( 2.699999999999946443, 2.500000000000000000, 0.3464101615137735735 ) ) ;
#6837=DIRECTION ( 'NONE',  ( 0.000000000000000000, 1.000000000000000000, 0.000000000000000000 ) ) ;
#6838=CARTESIAN_POINT ( 'NONE',  ( 9.999999999999948486, 12.50000000000000000, -4.330127018922201643 ) ) ;
#6839=LINE ( 'NONE', #78205, #16714 ) ;
#6840=AXIS2_PLACEMENT_3D ( 'NONE', #100128, #60844, #10447 ) ;
#6841=EDGE_CURVE ( 'NONE', #36786, #114224, #43043, .T. ) ;
#6842=DIRECTION ( 'NONE',  ( 0.000000000000000000, 0.000000000000000000, 1.000000000000000000 ) ) ;
#6843=AXIS2_PLACEMENT_3D ( 'NONE', #68652, #9735, #60148 ) ;
#6844=ORIENTED_EDGE ( 'NONE', *, *, #79714, .T. ) ;
#6845=AXIS2_PLACEMENT_3D ( 'NONE', #122552, #32895, #17722 ) ;
#6846=AXIS2_PLACEMENT_3D ( 'NONE', #80619, #68850, #89780 ) ;
#6847=FACE_OUTER_BOUND ( 'NONE', #65928, .T. ) ;
#6848=CARTESIAN_POINT ( 'NONE',  ( 12.69999999999989804, 2.500000000000000000, 0.3464101615137735735 ) ) ;
#6849=AXIS2_PLACEMENT_3D ( 'NONE', #100121, #60215, #38644 ) ;
#6850=ORIENTED_EDGE ( 'NONE', *, *, #79145, .F. ) ;
#6851=DIRECTION ( 'NONE',  ( -4.274815082592931898E-19, -0.9999939076577903929, -0.003490651415223739937 ) ) ;
#6852=ORIENTED_EDGE ( 'NONE', *, *, #125936, .T. ) ;
#6853=AXIS2_PLACEMENT_3D ( 'NONE', #91508, #102607, #23398 ) ;
#6855=ORIENTED_EDGE ( 'NONE', *, *, #65579, .T. ) ;
#6856=CARTESIAN_POINT ( 'NONE',  ( -7.100000000000017408, 2.500000000000000000, -5.022947341949754119 ) ) ;
#6857=AXIS2_PLACEMENT_3D ( 'NONE', #50246, #109135, #69215 ) ;
#6858=ORIENTED_EDGE ( 'NONE', *, *, #51244, .T. ) ;
#6859=CARTESIAN_POINT ( 'NONE',  ( -8.950000000000008171, 2.500000000000000000, 1.718653347947321386 ) ) ;
#6860=DIRECTION ( 'NONE',  ( 0.000000000000000000, 0.000000000000000000, 1.000000000000000000 ) ) ;
#6861=CARTESIAN_POINT ( 'NONE',  ( -8.150000000000012790, 2.500000000000000000, 2.611473670974873151 ) ) ;
#6862=VERTEX_POINT ( 'NONE', #89696 ) ;
#6863=FACE_BOUND ( 'NONE', #34324, .T. ) ;
#6864=AXIS2_PLACEMENT_3D ( 'NONE', #98688, #106585, #9025 ) ;
#6865=DIRECTION ( 'NONE',  ( 0.000000000000000000, 0.000000000000000000, -1.000000000000000000 ) ) ;
#6866=EDGE_LOOP ( 'NONE', ( #69901, #116492, #50831, #43463 ) ) ;
#6867=FACE_OUTER_BOUND ( 'NONE', #41202, .T. ) ;
#6869=VERTEX_POINT ( 'NONE', #30151 ) ;
#6870=ADVANCED_FACE ( 'NONE', ( #61539 ), #59621, .T. ) ;
#6871=ORIENTED_EDGE ( 'NONE', *, *, #490, .F. ) ;
#6872=EDGE_CURVE ( 'NONE', #125434, #120460, #11704, .T. ) ;
#6873=EDGE_LOOP ( 'NONE', ( #115402, #58640 ) ) ;
#6874=DIRECTION ( 'NONE',  ( 0.000000000000000000, 0.000000000000000000, -1.000000000000000000 ) ) ;
#6875=DIRECTION ( 'NONE',  ( 0.000000000000000000, 0.000000000000000000, 1.000000000000000000 ) ) ;
#6876=CONICAL_SURFACE ( 'NONE', #15201, 0.09999999999999982514, 0.003490658503988666988 ) ;
#6877=CARTESIAN_POINT ( 'NONE',  ( 0.4499999999999569344, 12.50000000000000000, 2.230156782645134950 ) ) ;
#6878=AXIS2_PLACEMENT_3D ( 'NONE', #68679, #27450, #67358 ) ;
#6879=FACE_BOUND ( 'NONE', #13108, .T. ) ;
#6880=ORIENTED_EDGE ( 'NONE', *, *, #48913, .F. ) ;
#6881=DIRECTION ( 'NONE',  ( -0.000000000000000000, -1.000000000000000000, -0.000000000000000000 ) ) ;
#6882=DIRECTION ( 'NONE',  ( 0.000000000000000000, 0.000000000000000000, 1.000000000000000000 ) ) ;
#6884=CONICAL_SURFACE ( 'NONE', #13152, 0.09999999999999982514, 0.003490658503988666988 ) ;
#6885=LINE ( 'NONE', #76308, #90973 ) ;
#6887=VECTOR ( 'NONE', #87608, 1000.000000000000000 ) ;
#6888=CARTESIAN_POINT ( 'NONE',  ( -4.400000000000025224, 2.500000000000000000, 0.4464101615137735513 ) ) ;
#6889=CIRCLE ( 'NONE', #25698, 0.06509327318403745899 ) ;
#6890=DIRECTION ( 'NONE',  ( 0.000000000000000000, -0.000000000000000000, 1.000000000000000000 ) ) ;
#6891=CARTESIAN_POINT ( 'NONE',  ( 1.649999999999950617, 12.50000000000000000, -2.230156782645139391 ) ) ;
#6892=DIRECTION ( 'NONE',  ( 0.000000000000000000, 0.000000000000000000, -1.000000000000000000 ) ) ;
#6893=VECTOR ( 'NONE', #42296, 1000.000000000000000 ) ;
#6895=ORIENTED_EDGE ( 'NONE', *, *, #17643, .T. ) ;
#6896=ORIENTED_EDGE ( 'NONE', *, *, #95147, .T. ) ;
#6897=EDGE_LOOP ( 'NONE', ( #121186, #123526 ) ) ;
#6898=ORIENTED_EDGE ( 'NONE', *, *, #68787, .T. ) ;
#6899=AXIS2_PLACEMENT_3D ( 'NONE', #105166, #55433, #115624 ) ;
#6900=ORIENTED_EDGE ( 'NONE', *, *, #100584, .T. ) ;
#6901=DIRECTION ( 'NONE',  ( -0.000000000000000000, -1.000000000000000000, -0.000000000000000000 ) ) ;
#6902=AXIS2_PLACEMENT_3D ( 'NONE', #25668, #47262, #48541 ) ;
#6903=CARTESIAN_POINT ( 'NONE',  ( 1.249999999999954259, 2.500000000000000000, -7.088010851410853519 ) ) ;
#6904=ORIENTED_EDGE ( 'NONE', *, *, #29176, .T. ) ;
#6905=FACE_BOUND ( 'NONE', #94056, .T. ) ;
#6906=CONICAL_SURFACE ( 'NONE', #107282, 0.1000000000000002554, 0.003490658503988666988 ) ;
#6907=DIRECTION ( 'NONE',  ( 0.000000000000000000, 1.000000000000000000, 0.000000000000000000 ) ) ;
#6908=LINE ( 'NONE', #16729, #999 ) ;
#6909=PLANE ( 'NONE',  #103840 ) ;
#6910=CARTESIAN_POINT ( 'NONE',  ( -3.150000000000029665, 2.500000000000000000, 6.941600689897073018 ) ) ;
#6911=DIRECTION ( 'NONE',  ( 0.000000000000000000, -0.9999939076577903929, 0.003490651415223739937 ) ) ;
#6912=ORIENTED_EDGE ( 'NONE', *, *, #22092, .T. ) ;
#6913=PLANE ( 'NONE',  #82755 ) ;
#6914=VECTOR ( 'NONE', #60987, 1000.000000000000000 ) ;
#6915=ORIENTED_EDGE ( 'NONE', *, *, #48209, .T. ) ;
#6917=ORIENTED_EDGE ( 'NONE', *, *, #34342, .T. ) ;
#6918=CARTESIAN_POINT ( 'NONE',  ( -8.300000000000009592, 12.50000000000000000, 4.330127018922196314 ) ) ;
#6919=FACE_OUTER_BOUND ( 'NONE', #74764, .T. ) ;
#6920=PLANE ( 'NONE',  #101163 ) ;
#6921=ORIENTED_EDGE ( 'NONE', *, *, #37486, .F. ) ;
#6922=CARTESIAN_POINT ( 'NONE',  ( 10.04522989421396417, 2.499999999999999556, -8.164691043410849502 ) ) ;
#6923=AXIS2_PLACEMENT_3D ( 'NONE', #128112, #37794, #58727 ) ;
#6924=AXIS2_PLACEMENT_3D ( 'NONE', #83408, #12698, #102399 ) ;
#6925=VECTOR ( 'NONE', #90765, 1000.000000000000000 ) ;
#6926=DIRECTION ( 'NONE',  ( -4.274815082592931898E-19, -0.9999939076577903929, -0.003490651415223739937 ) ) ;
#6927=CARTESIAN_POINT ( 'NONE',  ( -4.150000000000024336, 2.500000000000000000, 2.165063509461097713 ) ) ;
#6929=DIRECTION ( 'NONE',  ( -0.000000000000000000, 1.000000000000000000, -0.000000000000000000 ) ) ;
#6930=CARTESIAN_POINT ( 'NONE',  ( -9.150000000000009237, 12.50000000000000000, 2.857883832488649301 ) ) ;
#6931=ADVANCED_FACE ( 'NONE', ( #92260 ), #2583, .T. ) ;
#6932=CARTESIAN_POINT ( 'NONE',  ( 8.749999999999923617, 2.500000000000000000, 1.472243186433545459 ) ) ;
#6933=EDGE_CURVE ( 'NONE', #95501, #76430, #41262, .T. ) ;
#6934=CIRCLE ( 'NONE', #42587, 0.06509327318403745899 ) ;
#6935=ORIENTED_EDGE ( 'NONE', *, *, #8471, .T. ) ;
#6936=LINE ( 'NONE', #127394, #88099 ) ;
#6937=ORIENTED_EDGE ( 'NONE', *, *, #112797, .T. ) ;
#6938=CONICAL_SURFACE ( 'NONE', #4895, 0.1000000000000002554, 0.003490658503988666988 ) ;
#6939=EDGE_LOOP ( 'NONE', ( #77915, #97773, #93984, #54452 ) ) ;
#6940=DIRECTION ( 'NONE',  ( 0.000000000000000000, 0.000000000000000000, 1.000000000000000000 ) ) ;
#6941=DIRECTION ( 'NONE',  ( 0.000000000000000000, 0.000000000000000000, -1.000000000000000000 ) ) ;
#6942=PLANE ( 'NONE',  #119892 ) ;
#6943=ADVANCED_FACE ( 'NONE', ( #60877 ), #30519, .T. ) ;
#6944=ORIENTED_EDGE ( 'NONE', *, *, #115060, .F. ) ;
#6945=ORIENTED_EDGE ( 'NONE', *, *, #50269, .T. ) ;
#6946=LINE ( 'NONE', #56695, #1612 ) ;
#6947=FACE_OUTER_BOUND ( 'NONE', #4221, .T. ) ;
#6948=CIRCLE ( 'NONE', #113595, 0.06509327318403745899 ) ;
#6949=AXIS2_PLACEMENT_3D ( 'NONE', #94567, #105697, #55303 ) ;
#6950=AXIS2_PLACEMENT_3D ( 'NONE', #10964, #12899, #22129 ) ;
#6951=CARTESIAN_POINT ( 'NONE',  ( 8.149999999999920419, 2.500000000000000000, -1.818653347947325916 ) ) ;
#6952=ORIENTED_EDGE ( 'NONE', *, *, #39830, .F. ) ;
#6953=ORIENTED_EDGE ( 'NONE', *, *, #99648, .T. ) ;
#6954=CARTESIAN_POINT ( 'NONE',  ( -5.800000000000018474, 2.500000000000000000, 4.430127018922196847 ) ) ;
#6955=AXIS2_PLACEMENT_3D ( 'NONE', #116869, #107052, #48154 ) ;
#6956=EDGE_LOOP ( 'NONE', ( #44316, #11865, #36966, #39751 ) ) ;
#6957=DIRECTION ( 'NONE',  ( 0.000000000000000000, 0.000000000000000000, -1.000000000000000000 ) ) ;
#6958=FACE_OUTER_BOUND ( 'NONE', #111752, .T. ) ;
#6959=ORIENTED_EDGE ( 'NONE', *, *, #4945, .T. ) ;
#6960=DIRECTION ( 'NONE',  ( 0.000000000000000000, 1.000000000000000000, 0.000000000000000000 ) ) ;
#6961=EDGE_CURVE ( 'NONE', #9598, #2580, #128728, .T. ) ;
#6962=CARTESIAN_POINT ( 'NONE',  ( -9.200000000000006395, 2.500000000000000000, -2.385244779468109755E-15 ) ) ;
#6963=CARTESIAN_POINT ( 'NONE',  ( 5.399999999999936406, 2.500000000000000000, -3.537306695894649966 ) ) ;
#6964=DIRECTION ( 'NONE',  ( -4.274815082592931898E-19, -0.9999939076577903929, -0.003490651415223739937 ) ) ;
#6966=EDGE_CURVE ( 'NONE', #71302, #76450, #20, .T. ) ;
#6967=DIRECTION ( 'NONE',  ( 0.000000000000000000, 1.000000000000000000, 0.000000000000000000 ) ) ;
#6968=CARTESIAN_POINT ( 'NONE',  ( -3.750000000000027978, 12.50000000000000000, 7.188010851410848723 ) ) ;
#6969=ORIENTED_EDGE ( 'NONE', *, *, #69043, .T. ) ;
#6970=ORIENTED_EDGE ( 'NONE', *, *, #29345, .F. ) ;
#6971=EDGE_CURVE ( 'NONE', #37002, #122488, #84864, .T. ) ;
#6972=CIRCLE ( 'NONE', #19518, 0.06509327318403745899 ) ;
#6975=DIRECTION ( 'NONE',  ( 0.000000000000000000, 0.000000000000000000, 1.000000000000000000 ) ) ;
#6976=DIRECTION ( 'NONE',  ( -4.274815082592931898E-19, -0.9999939076577903929, -0.003490651415223739937 ) ) ;
#6977=EDGE_CURVE ( 'NONE', #78871, #72078, #47228, .T. ) ;
#6978=LINE ( 'NONE', #18754, #77216 ) ;
#6979=EDGE_CURVE ( 'NONE', #62883, #1523, #81170, .T. ) ;
#6980=PLANE ( 'NONE',  #105485 ) ;
#6981=DIRECTION ( 'NONE',  ( 0.000000000000000000, 1.000000000000000000, 0.000000000000000000 ) ) ;
#6982=AXIS2_PLACEMENT_3D ( 'NONE', #65796, #14740, #5575 ) ;
#6984=DIRECTION ( 'NONE',  ( 0.000000000000000000, 1.000000000000000000, 0.000000000000000000 ) ) ;
#6985=CONICAL_SURFACE ( 'NONE', #78126, 0.09999999999999999167, 0.003490658503988666988 ) ;
#6986=CARTESIAN_POINT ( 'NONE',  ( 2.499999999999945377, 12.50000000000000000, 5.022947341949748790 ) ) ;
#6987=DIRECTION ( 'NONE',  ( -0.000000000000000000, 1.000000000000000000, -0.000000000000000000 ) ) ;
#6988=CONICAL_SURFACE ( 'NONE', #92694, 0.1000000000000002554, 0.003490658503988666988 ) ;
#6989=EDGE_CURVE ( 'NONE', #34015, #116265, #63944, .T. ) ;
#6990=AXIS2_PLACEMENT_3D ( 'NONE', #129231, #17953, #78180 ) ;
#6991=ADVANCED_FACE ( 'NONE', ( #1309 ), #124582, .T. ) ;
#6992=LINE ( 'NONE', #87491, #73125 ) ;
#6993=VECTOR ( 'NONE', #52426, 1000.000000000000000 ) ;
#6994=AXIS2_PLACEMENT_3D ( 'NONE', #52120, #87921, #80062 ) ;
#6997=EDGE_LOOP ( 'NONE', ( #55547, #1217 ) ) ;
#6998=VECTOR ( 'NONE', #39047, 1000.000000000000000 ) ;
#6999=FACE_OUTER_BOUND ( 'NONE', #81090, .T. ) ;
#7000=CONICAL_SURFACE ( 'NONE', #15411, 0.09999999999999982514, 0.003490658503988666988 ) ;
#7001=VERTEX_POINT ( 'NONE', #34004 ) ;
#7003=DIRECTION ( 'NONE',  ( 0.000000000000000000, 0.000000000000000000, -1.000000000000000000 ) ) ;
#7004=DIRECTION ( 'NONE',  ( 0.000000000000000000, 1.000000000000000000, 0.000000000000000000 ) ) ;
#7005=DIRECTION ( 'NONE',  ( 0.000000000000000000, -0.9999939076577903929, 0.003490651415223739937 ) ) ;
#7006=EDGE_CURVE ( 'NONE', #91287, #2089, #34667, .T. ) ;
#7007=ORIENTED_EDGE ( 'NONE', *, *, #112535, .T. ) ;
#7008=LINE ( 'NONE', #54828, #96796 ) ;
#7009=DIRECTION ( 'NONE',  ( -0.000000000000000000, -1.000000000000000000, -0.000000000000000000 ) ) ;
#7010=CARTESIAN_POINT ( 'NONE',  ( 97.50000000000000000, -1.500000000000000222, -1.322875655532295136 ) ) ;
#7011=ORIENTED_EDGE ( 'NONE', *, *, #71151, .T. ) ;
#7012=AXIS2_PLACEMENT_3D ( 'NONE', #36705, #47807, #16373 ) ;
#7013=DIRECTION ( 'NONE',  ( -0.000000000000000000, 1.000000000000000000, -0.000000000000000000 ) ) ;
#7014=ORIENTED_EDGE ( 'NONE', *, *, #113076, .F. ) ;
#7015=EDGE_LOOP ( 'NONE', ( #103845, #126622 ) ) ;
#7016=EDGE_LOOP ( 'NONE', ( #15025, #40705, #49606, #68569 ) ) ;
#7017=VERTEX_POINT ( 'NONE', #23525 ) ;
#7018=CARTESIAN_POINT ( 'NONE',  ( -8.100000000000013856, 12.50000000000000000, -4.676537180435977881 ) ) ;
#7019=VECTOR ( 'NONE', #63235, 1000.000000000000000 ) ;
#7020=DIRECTION ( 'NONE',  ( 0.000000000000000000, 0.000000000000000000, 1.000000000000000000 ) ) ;
#7021=DIRECTION ( 'NONE',  ( 0.000000000000000000, -0.000000000000000000, 1.000000000000000000 ) ) ;
#7022=AXIS2_PLACEMENT_3D ( 'NONE', #52480, #119947, #102859 ) ;
#7023=LINE ( 'NONE', #128114, #120935 ) ;
#7024=AXIS2_PLACEMENT_3D ( 'NONE', #76288, #113636, #36384 ) ;
#7025=ORIENTED_EDGE ( 'NONE', *, *, #61176, .T. ) ;
#7026=DIRECTION ( 'NONE',  ( 0.000000000000000000, 1.000000000000000000, 0.000000000000000000 ) ) ;
#7027=ORIENTED_EDGE ( 'NONE', *, *, #19449, .F. ) ;
#7028=CARTESIAN_POINT ( 'NONE',  ( 12.49999999999990052, 2.500000000000000000, 0.6928203230275494784 ) ) ;
#7029=CARTESIAN_POINT ( 'NONE',  ( -2.100000000000033396, 2.500000000000000000, -0.7928203230275543412 ) ) ;
#7030=DIRECTION ( 'NONE',  ( -4.274815082592931898E-19, -0.9999939076577903929, -0.003490651415223739937 ) ) ;
#7031=DIRECTION ( 'NONE',  ( -0.000000000000000000, -1.000000000000000000, -0.000000000000000000 ) ) ;
#7032=VECTOR ( 'NONE', #71144, 1000.000000000000000 ) ;
#7033=VECTOR ( 'NONE', #9580, 1000.000000000000000 ) ;
#7034=AXIS2_PLACEMENT_3D ( 'NONE', #40964, #79578, #120781 ) ;
#7035=ORIENTED_EDGE ( 'NONE', *, *, #19450, .F. ) ;
#7036=VECTOR ( 'NONE', #81573, 1000.000000000000000 ) ;
#7037=EDGE_CURVE ( 'NONE', #19146, #30332, #53640, .T. ) ;
#7038=VERTEX_POINT ( 'NONE', #92933 ) ;
#7039=VERTEX_POINT ( 'NONE', #124960 ) ;
#7040=EDGE_CURVE ( 'NONE', #53498, #128103, #22197, .T. ) ;
#7041=ORIENTED_EDGE ( 'NONE', *, *, #55143, .F. ) ;
#7042=DIRECTION ( 'NONE',  ( -0.000000000000000000, -1.000000000000000000, -0.000000000000000000 ) ) ;
#7043=CARTESIAN_POINT ( 'NONE',  ( 76.44836599003085098, 3.583082429763411625, 6.086789565880034836 ) ) ;
#7044=DIRECTION ( 'NONE',  ( 0.000000000000000000, 0.000000000000000000, 1.000000000000000000 ) ) ;
#7045=FACE_BOUND ( 'NONE', #106291, .T. ) ;
#7046=AXIS2_PLACEMENT_3D ( 'NONE', #89387, #20008, #129334 ) ;
#7047=DIRECTION ( 'NONE',  ( -0.000000000000000000, 1.000000000000000000, -0.000000000000000000 ) ) ;
#7048=CARTESIAN_POINT ( 'NONE',  ( 9.149999999999916866, 12.50000000000000000, 7.188010851410848723 ) ) ;
#7049=DIRECTION ( 'NONE',  ( 0.000000000000000000, 0.000000000000000000, -1.000000000000000000 ) ) ;
#7050=DIRECTION ( 'NONE',  ( 0.000000000000000000, 0.000000000000000000, 1.000000000000000000 ) ) ;
#7051=CIRCLE ( 'NONE', #48944, 0.1000000000000002554 ) ;
#7052=AXIS2_PLACEMENT_3D ( 'NONE', #51936, #2170, #7893 ) ;
#7053=CIRCLE ( 'NONE', #4910, 0.06509327318403745899 ) ;
#7055=DIRECTION ( 'NONE',  ( 0.000000000000000000, 1.000000000000000000, 0.000000000000000000 ) ) ;
#7056=CIRCLE ( 'NONE', #94909, 0.06509327318403745899 ) ;
#7057=DIRECTION ( 'NONE',  ( 0.000000000000000000, 0.000000000000000000, 1.000000000000000000 ) ) ;
#7058=AXIS2_PLACEMENT_3D ( 'NONE', #36230, #73549, #64384 ) ;
#7059=DIRECTION ( 'NONE',  ( 0.000000000000000000, 0.000000000000000000, -1.000000000000000000 ) ) ;
#7060=ORIENTED_EDGE ( 'NONE', *, *, #102567, .T. ) ;
#7062=ORIENTED_EDGE ( 'NONE', *, *, #2127, .T. ) ;
#7063=ORIENTED_EDGE ( 'NONE', *, *, #85580, .F. ) ;
#7064=CARTESIAN_POINT ( 'NONE',  ( -12.49999999999999289, 2.500000000000000000, -4.922947341949750921 ) ) ;
#7065=FACE_BOUND ( 'NONE', #104403, .T. ) ;
#7066=DIRECTION ( 'NONE',  ( -4.274815082592931898E-19, -0.9999939076577903929, -0.003490651415223739937 ) ) ;
#7067=CARTESIAN_POINT ( 'NONE',  ( 1.649999999999951505, 2.500000000000000000, 1.472243186433545459 ) ) ;
#7068=AXIS2_PLACEMENT_3D ( 'NONE', #113074, #52240, #41792 ) ;
#7069=ORIENTED_EDGE ( 'NONE', *, *, #12098, .F. ) ;
#7070=CARTESIAN_POINT ( 'NONE',  ( -3.550000000000027356, 2.500000000000000000, 1.918653347947321564 ) ) ;
#7071=AXIS2_PLACEMENT_3D ( 'NONE', #95490, #26112, #66024 ) ;
#7072=FACE_OUTER_BOUND ( 'NONE', #113542, .T. ) ;
#7073=VERTEX_POINT ( 'NONE', #24824 ) ;
#7074=CARTESIAN_POINT ( 'NONE',  ( 12.09999999999990550, 2.500000000000000000, 4.430127018922196847 ) ) ;
#7075=CARTESIAN_POINT ( 'NONE',  ( -4.400000000000025224, 2.500000000000000000, 3.883716857408420431 ) ) ;
#7076=EDGE_CURVE ( 'NONE', #50039, #44638, #95336, .T. ) ;
#7077=AXIS2_PLACEMENT_3D ( 'NONE', #120072, #30420, #101071 ) ;
#7078=CIRCLE ( 'NONE', #53077, 0.1000000000000002554 ) ;
#7079=VECTOR ( 'NONE', #11376, 1000.000000000000000 ) ;
#7080=AXIS2_PLACEMENT_3D ( 'NONE', #44162, #35017, #84078 ) ;
#7081=AXIS2_PLACEMENT_3D ( 'NONE', #81242, #11837, #60943 ) ;
#7082=EDGE_LOOP ( 'NONE', ( #44611, #5300, #22087, #124119 ) ) ;
#7083=PLANE ( 'NONE',  #73790 ) ;
#7084=DIRECTION ( 'NONE',  ( -0.000000000000000000, -1.000000000000000000, -0.000000000000000000 ) ) ;
#7085=EDGE_CURVE ( 'NONE', #22780, #21628, #44460, .T. ) ;
#7086=CIRCLE ( 'NONE', #128313, 0.06509327318403745899 ) ;
#7087=CIRCLE ( 'NONE', #42645, 0.06509327318403745899 ) ;
#7088=VERTEX_POINT ( 'NONE', #93568 ) ;
#7089=AXIS2_PLACEMENT_3D ( 'NONE', #81930, #73404, #13184 ) ;
#7090=CARTESIAN_POINT ( 'NONE',  ( 2.049999999999948308, 2.500000000000000000, 6.495190528383297135 ) ) ;
#7091=DIRECTION ( 'NONE',  ( 0.000000000000000000, 0.000000000000000000, 1.000000000000000000 ) ) ;
#7092=ORIENTED_EDGE ( 'NONE', *, *, #29012, .T. ) ;
#7093=CARTESIAN_POINT ( 'NONE',  ( -9.150000000000009237, 2.500000000000000000, 2.265063509461097357 ) ) ;
#7094=CIRCLE ( 'NONE', #117816, 0.06509327318403745899 ) ;
#7095=ORIENTED_EDGE ( 'NONE', *, *, #10518, .T. ) ;
#7097=VERTEX_POINT ( 'NONE', #113855 ) ;
#7098=EDGE_CURVE ( 'NONE', #104335, #48350, #51521, .T. ) ;
#7099=CARTESIAN_POINT ( 'NONE',  ( 5.399999999999934630, 2.500000000000000000, 0.6928203230275494784 ) ) ;
#7100=VERTEX_POINT ( 'NONE', #13699 ) ;
#7101=DIRECTION ( 'NONE',  ( 0.000000000000000000, 0.000000000000000000, 1.000000000000000000 ) ) ;
#7102=CARTESIAN_POINT ( 'NONE',  ( 3.299999999999944755, 12.50000000000000000, 0.06509327318403504425 ) ) ;
#7103=ORIENTED_EDGE ( 'NONE', *, *, #85728, .F. ) ;
#7104=DIRECTION ( 'NONE',  ( 0.000000000000000000, 1.000000000000000000, 0.000000000000000000 ) ) ;
#7105=ORIENTED_EDGE ( 'NONE', *, *, #63345, .F. ) ;
#7106=DIRECTION ( 'NONE',  ( -0.000000000000000000, 1.000000000000000000, -0.000000000000000000 ) ) ;
#7107=AXIS2_PLACEMENT_3D ( 'NONE', #33848, #92116, #102580 ) ;
#7108=CARTESIAN_POINT ( 'NONE',  ( -0.4000000000000401013, 2.500000000000000000, -3.637306695894650055 ) ) ;
#7109=FACE_OUTER_BOUND ( 'NONE', #4483, .T. ) ;
#7110=DIRECTION ( 'NONE',  ( -4.274815082592931898E-19, -0.9999939076577903929, -0.003490651415223739937 ) ) ;
#7111=EDGE_CURVE ( 'NONE', #2654, #79541, #45257, .T. ) ;
#7112=DIRECTION ( 'NONE',  ( 0.000000000000000000, -0.9999939076577903929, 0.003490651415223739937 ) ) ;
#7113=AXIS2_PLACEMENT_3D ( 'NONE', #88111, #85563, #37758 ) ;
#7114=VERTEX_POINT ( 'NONE', #73923 ) ;
#7115=VERTEX_POINT ( 'NONE', #115108 ) ;
#7116=FACE_OUTER_BOUND ( 'NONE', #59392, .T. ) ;
#7117=CARTESIAN_POINT ( 'NONE',  ( -12.89999999999999147, 2.500000000000000000, -4.330127018922198978 ) ) ;
#7118=DIRECTION ( 'NONE',  ( -4.274815082592931898E-19, -0.9999939076577903929, -0.003490651415223739937 ) ) ;
#7119=ORIENTED_EDGE ( 'NONE', *, *, #125365, .F. ) ;
#7120=EDGE_LOOP ( 'NONE', ( #74979, #122568 ) ) ;
#7121=ORIENTED_EDGE ( 'NONE', *, *, #32601, .F. ) ;
#7122=CARTESIAN_POINT ( 'NONE',  ( -6.650000000000018119, 12.50000000000000000, -2.230156782645139391 ) ) ;
#7123=CIRCLE ( 'NONE', #105439, 0.1000000000000002554 ) ;
#7124=CARTESIAN_POINT ( 'NONE',  ( -3.950000000000024603, 2.500000000000000000, -2.511473670974877948 ) ) ;
#7125=CIRCLE ( 'NONE', #36403, 0.1000000000000002554 ) ;
#7126=CARTESIAN_POINT ( 'NONE',  ( -13.94999999999998685, 2.500000000000000000, -2.411473670974875638 ) ) ;
#7127=CARTESIAN_POINT ( 'NONE',  ( 1.649999999999951505, 2.500000000000000000, 2.857883832488649301 ) ) ;
#7128=LINE ( 'NONE', #66059, #6285 ) ;
#7129=CARTESIAN_POINT ( 'NONE',  ( 0.8499999999999553468, 12.50000000000000000, 2.165063509461097713 ) ) ;
#7130=CARTESIAN_POINT ( 'NONE',  ( -8.150000000000014566, 2.500000000000000000, -6.841600689897073373 ) ) ;
#7131=CARTESIAN_POINT ( 'NONE',  ( -8.150000000000014566, 12.50000000000000000, -6.148780366869520897 ) ) ;
#7132=DIRECTION ( 'NONE',  ( 0.000000000000000000, 0.000000000000000000, 1.000000000000000000 ) ) ;
#7133=EDGE_LOOP ( 'NONE', ( #41566, #109180, #41717, #80305 ) ) ;
#7134=CIRCLE ( 'NONE', #21843, 0.06509327318403745899 ) ;
#7135=ADVANCED_FACE ( 'NONE', ( #3886 ), #43844, .T. ) ;
#7136=DIRECTION ( 'NONE',  ( 0.000000000000000000, 0.000000000000000000, -1.000000000000000000 ) ) ;
#7137=ORIENTED_EDGE ( 'NONE', *, *, #119319, .F. ) ;
#7138=VERTEX_POINT ( 'NONE', #104033 ) ;
#7139=EDGE_CURVE ( 'NONE', #129332, #78385, #14339, .T. ) ;
#7140=DIRECTION ( 'NONE',  ( -0.000000000000000000, 1.000000000000000000, -0.000000000000000000 ) ) ;
#7141=CARTESIAN_POINT ( 'NONE',  ( 15.19999999999989271, 12.50000000000000000, -0.2813168883297409439 ) ) ;
#7142=DIRECTION ( 'NONE',  ( 0.000000000000000000, 0.000000000000000000, -1.000000000000000000 ) ) ;
#7143=ADVANCED_FACE ( 'NONE', ( #74568 ), #53576, .T. ) ;
#7144=CARTESIAN_POINT ( 'NONE',  ( -13.14999999999999147, 12.50000000000000000, 2.511473670974877503 ) ) ;
#7145=DIRECTION ( 'NONE',  ( 0.000000000000000000, 0.000000000000000000, 1.000000000000000000 ) ) ;
#7146=VECTOR ( 'NONE', #74686, 1000.000000000000000 ) ;
#7147=DIRECTION ( 'NONE',  ( 0.000000000000000000, 0.000000000000000000, 1.000000000000000000 ) ) ;
#7148=AXIS2_PLACEMENT_3D ( 'NONE', #9321, #79367, #30274 ) ;
#7149=CARTESIAN_POINT ( 'NONE',  ( 14.34999999999989306, 2.500000000000000000, -2.611473670974877592 ) ) ;
#7150=ORIENTED_EDGE ( 'NONE', *, *, #91105, .T. ) ;
#7151=CARTESIAN_POINT ( 'NONE',  ( 1.049999999999953637, 2.500000000000000000, 2.511473670974873507 ) ) ;
#7152=ADVANCED_FACE ( 'NONE', ( #95496 ), #76558, .T. ) ;
#7153=ADVANCED_FACE ( 'NONE', ( #115778 ), #105962, .T. ) ;
#7154=CONICAL_SURFACE ( 'NONE', #82494, 0.1000000000000002554, 0.003490658503988666988 ) ;
#7155=ADVANCED_FACE ( 'NONE', ( #75843 ), #93281, .T. ) ;
#7156=ADVANCED_FACE ( 'NONE', ( #27378 ), #128814, .T. ) ;
#7157=AXIS2_PLACEMENT_3D ( 'NONE', #57468, #87553, #50233 ) ;
#7158=DIRECTION ( 'NONE',  ( -4.274815082592931898E-19, -0.9999939076577903929, -0.003490651415223739937 ) ) ;
#7159=ORIENTED_EDGE ( 'NONE', *, *, #43555, .F. ) ;
#7160=ADVANCED_FACE ( 'NONE', ( #18859 ), #15897, .T. ) ;
#7162=VERTEX_POINT ( 'NONE', #97421 ) ;
#7163=ORIENTED_EDGE ( 'NONE', *, *, #36078, .T. ) ;
#7164=LINE ( 'NONE', #108601, #46199 ) ;
#7165=DIRECTION ( 'NONE',  ( 0.000000000000000000, 1.000000000000000000, 0.000000000000000000 ) ) ;
#7167=EDGE_LOOP ( 'NONE', ( #44695, #53554, #64970, #4318 ) ) ;
#7168=DIRECTION ( 'NONE',  ( 0.000000000000000000, 0.000000000000000000, 1.000000000000000000 ) ) ;
#7169=DIRECTION ( 'NONE',  ( 0.000000000000000000, 1.000000000000000000, 0.000000000000000000 ) ) ;
#7170=CONICAL_SURFACE ( 'NONE', #101271, 0.1000000000000002554, 0.003490658503988666988 ) ;
#7171=AXIS2_PLACEMENT_3D ( 'NONE', #55472, #6331, #116301 ) ;
#7172=CARTESIAN_POINT ( 'NONE',  ( 7.299999999999926104, 2.500000000000000000, -3.883716857408426648 ) ) ;
#7173=EDGE_LOOP ( 'NONE', ( #34390, #39269 ) ) ;
#7175=VECTOR ( 'NONE', #75057, 1000.000000000000000 ) ;
#7176=DIRECTION ( 'NONE',  ( 0.000000000000000000, 0.000000000000000000, 1.000000000000000000 ) ) ;
#7178=ORIENTED_EDGE ( 'NONE', *, *, #16275, .T. ) ;
#7179=VECTOR ( 'NONE', #9309, 1000.000000000000000 ) ;
#7180=CONICAL_SURFACE ( 'NONE', #23934, 0.1000000000000002554, 0.003490658503988666988 ) ;
#7181=VERTEX_POINT ( 'NONE', #58800 ) ;
#7182=EDGE_LOOP ( 'NONE', ( #85221, #123465, #97254, #129422 ) ) ;
#7183=CARTESIAN_POINT ( 'NONE',  ( 4.799999999999934097, 2.500000000000000000, 4.676537180435972552 ) ) ;
#7184=CARTESIAN_POINT ( 'NONE',  ( -1.650000000000035660, 12.50000000000000000, 7.122917578226811486 ) ) ;
#7185=CONICAL_SURFACE ( 'NONE', #9262, 0.1000000000000000472, 0.003490658503988666988 ) ;
#7186=AXIS2_PLACEMENT_3D ( 'NONE', #5787, #46365, #26739 ) ;
#7187=VECTOR ( 'NONE', #121622, 1000.000000000000000 ) ;
#7188=ORIENTED_EDGE ( 'NONE', *, *, #38743, .T. ) ;
#7189=DIRECTION ( 'NONE',  ( -4.274815082592931898E-19, -0.9999939076577903929, -0.003490651415223739937 ) ) ;
#7190=CARTESIAN_POINT ( 'NONE',  ( -9.200000000000006395, 12.50000000000000000, 4.265033745738159077 ) ) ;
#7191=DIRECTION ( 'NONE',  ( -0.000000000000000000, -1.000000000000000000, -0.000000000000000000 ) ) ;
#7192=DIRECTION ( 'NONE',  ( -0.000000000000000000, -1.000000000000000000, -0.000000000000000000 ) ) ;
#7193=ORIENTED_EDGE ( 'NONE', *, *, #97659, .T. ) ;
#7194=DIRECTION ( 'NONE',  ( -0.000000000000000000, 1.000000000000000000, -0.000000000000000000 ) ) ;
#7195=ADVANCED_FACE ( 'NONE', ( #98066 ), #18212, .T. ) ;
#7196=ORIENTED_EDGE ( 'NONE', *, *, #64781, .F. ) ;
#7197=ORIENTED_EDGE ( 'NONE', *, *, #28903, .F. ) ;
#7198=ORIENTED_EDGE ( 'NONE', *, *, #32344, .F. ) ;
#7199=DIRECTION ( 'NONE',  ( 0.000000000000000000, 1.000000000000000000, 0.000000000000000000 ) ) ;
#7200=FACE_BOUND ( 'NONE', #63566, .T. ) ;
#7201=LINE ( 'NONE', #47800, #22122 ) ;
#7202=AXIS2_PLACEMENT_3D ( 'NONE', #65692, #16573, #77448 ) ;
#7203=CARTESIAN_POINT ( 'NONE',  ( 14.14999999999989555, 2.500000000000000000, 2.165063509461097713 ) ) ;
#7204=DIRECTION ( 'NONE',  ( -0.000000000000000000, 1.000000000000000000, -0.000000000000000000 ) ) ;
#7205=EDGE_CURVE ( 'NONE', #41083, #87429, #47310, .T. ) ;
#7206=ORIENTED_EDGE ( 'NONE', *, *, #2807, .T. ) ;
#7207=CARTESIAN_POINT ( 'NONE',  ( 11.24999999999990763, 2.500000000000000000, -7.188010851410854052 ) ) ;
#7208=CARTESIAN_POINT ( 'NONE',  ( -6.650000000000018119, 12.50000000000000000, -7.253104124594891289 ) ) ;
#7209=CARTESIAN_POINT ( 'NONE',  ( 17.49862860983209956, 2.500000000000000000, 4.081131818001135336 ) ) ;
#7210=DIRECTION ( 'NONE',  ( 0.000000000000000000, 0.000000000000000000, 1.000000000000000000 ) ) ;
#7211=ORIENTED_EDGE ( 'NONE', *, *, #97695, .F. ) ;
#7212=VECTOR ( 'NONE', #12379, 1000.000000000000000 ) ;
#7214=DIRECTION ( 'NONE',  ( -0.000000000000000000, -1.000000000000000000, -0.000000000000000000 ) ) ;
#7215=ORIENTED_EDGE ( 'NONE', *, *, #12766, .F. ) ;
#7216=DIRECTION ( 'NONE',  ( 0.000000000000000000, 0.000000000000000000, -1.000000000000000000 ) ) ;
#7217=DIRECTION ( 'NONE',  ( 0.000000000000000000, 1.000000000000000000, 0.000000000000000000 ) ) ;
#7218=FACE_BOUND ( 'NONE', #72971, .T. ) ;
#7219=CARTESIAN_POINT ( 'NONE',  ( 12.89999999999990088, 2.500000000000000000, -4.330127018922201643 ) ) ;
#7220=AXIS2_PLACEMENT_3D ( 'NONE', #13960, #122001, #92527 ) ;
#7221=VERTEX_POINT ( 'NONE', #67283 ) ;
#7222=CARTESIAN_POINT ( 'NONE',  ( -14.39999999999998614, 12.50000000000000000, 0.3464101615137758494 ) ) ;
#7223=AXIS2_PLACEMENT_3D ( 'NONE', #119782, #27516, #117830 ) ;
#7224=ORIENTED_EDGE ( 'NONE', *, *, #58871, .T. ) ;
#7225=EDGE_LOOP ( 'NONE', ( #89757, #117652 ) ) ;
#7226=DIRECTION ( 'NONE',  ( 0.000000000000000000, -0.000000000000000000, 1.000000000000000000 ) ) ;
#7228=ORIENTED_EDGE ( 'NONE', *, *, #52058, .F. ) ;
#7230=DIRECTION ( 'NONE',  ( 0.000000000000000000, -0.9999939076577903929, 0.003490651415223739937 ) ) ;
#7231=EDGE_CURVE ( 'NONE', #35583, #102949, #9653, .T. ) ;
#7232=AXIS2_PLACEMENT_3D ( 'NONE', #79211, #98827, #18971 ) ;
#7234=LINE ( 'NONE', #63934, #101229 ) ;
#7235=CIRCLE ( 'NONE', #95096, 0.09999999999999982514 ) ;
#7237=AXIS2_PLACEMENT_3D ( 'NONE', #18011, #27190, #78249 ) ;
#7238=EDGE_CURVE ( 'NONE', #12542, #51573, #36853, .T. ) ;
#7239=ORIENTED_EDGE ( 'NONE', *, *, #71906, .F. ) ;
#7240=CARTESIAN_POINT ( 'NONE',  ( 8.149999999999920419, 2.500000000000000000, -2.511473670974877948 ) ) ;
#7241=CARTESIAN_POINT ( 'NONE',  ( 5.849999999999933031, 12.50000000000000000, 7.122917578226811486 ) ) ;
#7242=FACE_OUTER_BOUND ( 'NONE', #40721, .T. ) ;
#7243=CARTESIAN_POINT ( 'NONE',  ( 10.19999999999991225, 2.500000000000000000, 3.983716857408420076 ) ) ;
#7244=EDGE_LOOP ( 'NONE', ( #62942, #63922, #43575, #19900 ) ) ;
#7245=EDGE_CURVE ( 'NONE', #51302, #94018, #32670, .T. ) ;
#7246=DIRECTION ( 'NONE',  ( -0.000000000000000000, 1.000000000000000000, -0.000000000000000000 ) ) ;
#7247=ORIENTED_EDGE ( 'NONE', *, *, #79319, .T. ) ;
#7248=EDGE_CURVE ( 'NONE', #78678, #50948, #114211, .T. ) ;
#7249=DIRECTION ( 'NONE',  ( 0.000000000000000000, 1.000000000000000000, 0.000000000000000000 ) ) ;
#7250=CARTESIAN_POINT ( 'NONE',  ( 1.699999999999950218, 12.50000000000000000, 4.330127018922196314 ) ) ;
#7251=ORIENTED_EDGE ( 'NONE', *, *, #18073, .T. ) ;
#7252=FACE_OUTER_BOUND ( 'NONE', #45506, .T. ) ;
#7253=CARTESIAN_POINT ( 'NONE',  ( 10.44999999999991402, 2.500000000000000000, -2.065063509461102065 ) ) ;
#7254=DIRECTION ( 'NONE',  ( -0.000000000000000000, -1.000000000000000000, -0.000000000000000000 ) ) ;
#7255=AXIS2_PLACEMENT_3D ( 'NONE', #116462, #125636, #6480 ) ;
#7256=CARTESIAN_POINT ( 'NONE',  ( -4.350000000000023626, 12.50000000000000000, 6.841600689897072485 ) ) ;
#7257=ORIENTED_EDGE ( 'NONE', *, *, #65843, .T. ) ;
#7258=ADVANCED_FACE ( 'NONE', ( #76507 ), #122526, .T. ) ;
#7259=AXIS2_PLACEMENT_3D ( 'NONE', #18108, #40354, #28590 ) ;
#7260=CARTESIAN_POINT ( 'NONE',  ( 11.04999999999991012, 2.500000000000000000, -1.718653347947326049 ) ) ;
#7261=FACE_OUTER_BOUND ( 'NONE', #25716, .T. ) ;
#7262=AXIS2_PLACEMENT_3D ( 'NONE', #14702, #76236, #64463 ) ;
#7263=CIRCLE ( 'NONE', #118085, 0.06509327318403745899 ) ;
#7265=CARTESIAN_POINT ( 'NONE',  ( 7.899999999999924860, 2.500000000000000000, -4.330127018922201643 ) ) ;
#7266=EDGE_CURVE ( 'NONE', #9428, #93110, #103749, .T. ) ;
#7267=CARTESIAN_POINT ( 'NONE',  ( 5.849999999999935696, 2.500000000000000000, -6.595190528383302109 ) ) ;
#7268=CIRCLE ( 'NONE', #80462, 0.06509327318403741736 ) ;
#7269=EDGE_LOOP ( 'NONE', ( #61812, #5739 ) ) ;
#7270=EDGE_LOOP ( 'NONE', ( #122029, #46509 ) ) ;
#7271=CIRCLE ( 'NONE', #113908, 0.06509327318403745899 ) ;
#7272=CARTESIAN_POINT ( 'NONE',  ( 11.89999999999990443, 2.500000000000000000, -0.3464101615137782364 ) ) ;
#7273=ORIENTED_EDGE ( 'NONE', *, *, #121200, .F. ) ;
#7274=CARTESIAN_POINT ( 'NONE',  ( -14.59999999999998366, 2.500000000000000000, -1.084202172485504434E-16 ) ) ;
#7275=AXIS2_PLACEMENT_3D ( 'NONE', #119549, #61295, #109752 ) ;
#7276=ORIENTED_EDGE ( 'NONE', *, *, #96380, .T. ) ;
#7277=ORIENTED_EDGE ( 'NONE', *, *, #91362, .T. ) ;
#7278=ORIENTED_EDGE ( 'NONE', *, *, #129130, .F. ) ;
#7279=CARTESIAN_POINT ( 'NONE',  ( -15.39999999999997904, 2.500000000000000000, -0.1000000000000000056 ) ) ;
#7280=CIRCLE ( 'NONE', #21987, 0.1000000000000000472 ) ;
#7281=CARTESIAN_POINT ( 'NONE',  ( 6.449999999999928235, 12.50000000000000000, 2.511473670974873507 ) ) ;
#7282=CIRCLE ( 'NONE', #116049, 0.06509327318403745899 ) ;
#7283=DIRECTION ( 'NONE',  ( 0.000000000000000000, 0.000000000000000000, 1.000000000000000000 ) ) ;
#7284=CARTESIAN_POINT ( 'NONE',  ( 9.149999999999916866, 12.50000000000000000, -2.857883832488653741 ) ) ;
#7285=DIRECTION ( 'NONE',  ( 0.000000000000000000, 0.000000000000000000, 1.000000000000000000 ) ) ;
#7286=VECTOR ( 'NONE', #104566, 1000.000000000000000 ) ;
#7287=PLANE ( 'NONE',  #47651 ) ;
#7289=CARTESIAN_POINT ( 'NONE',  ( 13.29999999999990301, 2.500000000000000000, -4.430127018922202176 ) ) ;
#7290=ORIENTED_EDGE ( 'NONE', *, *, #74829, .T. ) ;
#7291=ORIENTED_EDGE ( 'NONE', *, *, #108108, .T. ) ;
#7292=ORIENTED_EDGE ( 'NONE', *, *, #83179, .T. ) ;
#7293=ORIENTED_EDGE ( 'NONE', *, *, #32181, .T. ) ;
#7294=DIRECTION ( 'NONE',  ( 0.000000000000000000, 0.000000000000000000, -1.000000000000000000 ) ) ;
#7295=ORIENTED_EDGE ( 'NONE', *, *, #36520, .T. ) ;
#7296=ORIENTED_EDGE ( 'NONE', *, *, #62355, .T. ) ;
#7297=AXIS2_PLACEMENT_3D ( 'NONE', #1456, #79395, #50554 ) ;
#7298=DIRECTION ( 'NONE',  ( 0.000000000000000000, 0.000000000000000000, 1.000000000000000000 ) ) ;
#7299=DIRECTION ( 'NONE',  ( -0.000000000000000000, 1.000000000000000000, -0.000000000000000000 ) ) ;
#7301=LINE ( 'NONE', #88442, #54654 ) ;
#7302=FACE_OUTER_BOUND ( 'NONE', #4448, .T. ) ;
#7303=ADVANCED_FACE ( 'NONE', ( #87596 ), #18048, .T. ) ;
#7304=DIRECTION ( 'NONE',  ( -0.000000000000000000, 1.000000000000000000, -0.000000000000000000 ) ) ;
#7305=EDGE_LOOP ( 'NONE', ( #122179, #105513 ) ) ;
#7306=EDGE_CURVE ( 'NONE', #71809, #104716, #97483, .T. ) ;
#7307=EDGE_CURVE ( 'NONE', #62993, #107468, #118407, .T. ) ;
#7308=DIRECTION ( 'NONE',  ( 0.000000000000000000, 0.000000000000000000, 1.000000000000000000 ) ) ;
#7309=AXIS2_PLACEMENT_3D ( 'NONE', #94517, #85350, #24500 ) ;
#7310=ADVANCED_FACE ( 'NONE', ( #38539 ), #3388, .T. ) ;
#7311=CIRCLE ( 'NONE', #95156, 0.09999999999999999167 ) ;
#7312=EDGE_LOOP ( 'NONE', ( #3928, #86218, #39468, #29700 ) ) ;
#7313=CARTESIAN_POINT ( 'NONE',  ( -1.050000000000037792, 12.50000000000000000, 6.213873640053558134 ) ) ;
#7314=ORIENTED_EDGE ( 'NONE', *, *, #50167, .T. ) ;
#7315=CARTESIAN_POINT ( 'NONE',  ( 11.44999999999990514, 2.500000000000000000, -6.148780366869526226 ) ) ;
#7316=ADVANCED_FACE ( 'NONE', ( #11622 ), #78715, .T. ) ;
#7317=ORIENTED_EDGE ( 'NONE', *, *, #57930, .T. ) ;
#7318=ORIENTED_EDGE ( 'NONE', *, *, #41614, .T. ) ;
#7319=DIRECTION ( 'NONE',  ( 0.000000000000000000, -0.9999939076577903929, 0.003490651415223739937 ) ) ;
#7320=DIRECTION ( 'NONE',  ( 0.000000000000000000, 0.000000000000000000, -1.000000000000000000 ) ) ;
#7321=ADVANCED_FACE ( 'NONE', ( #60735 ), #128906, .T. ) ;
#7322=AXIS2_PLACEMENT_3D ( 'NONE', #54377, #33474, #84496 ) ;
#7323=EDGE_CURVE ( 'NONE', #71326, #98343, #55706, .T. ) ;
#7324=DIRECTION ( 'NONE',  ( -4.274815082592931898E-19, -0.9999939076577903929, -0.003490651415223739937 ) ) ;
#7325=LINE ( 'NONE', #66891, #56973 ) ;
#7326=VECTOR ( 'NONE', #41246, 1000.000000000000000 ) ;
#7327=DIRECTION ( 'NONE',  ( 0.000000000000000000, 1.000000000000000000, 0.000000000000000000 ) ) ;
#7329=FACE_OUTER_BOUND ( 'NONE', #7754, .T. ) ;
#7330=DIRECTION ( 'NONE',  ( -0.000000000000000000, -1.000000000000000000, -0.000000000000000000 ) ) ;
#7331=CARTESIAN_POINT ( 'NONE',  ( -10.80000000000000071, 2.500000000000000000, 4.330127018922196314 ) ) ;
#7332=CARTESIAN_POINT ( 'NONE',  ( -0.4500000000000397571, 12.50000000000000000, -6.560283801567339701 ) ) ;
#7333=CARTESIAN_POINT ( 'NONE',  ( 2.699999999999944666, 2.500000000000000000, 4.576537180435972019 ) ) ;
#7334=ORIENTED_EDGE ( 'NONE', *, *, #80756, .T. ) ;
#7335=AXIS2_PLACEMENT_3D ( 'NONE', #95942, #67768, #46194 ) ;
#7336=AXIS2_PLACEMENT_3D ( 'NONE', #71659, #61199, #101122 ) ;
#7337=EDGE_LOOP ( 'NONE', ( #95649, #81461, #7692, #112398 ) ) ;
#7338=FACE_OUTER_BOUND ( 'NONE', #117262, .T. ) ;
#7339=EDGE_CURVE ( 'NONE', #40266, #55057, #66082, .T. ) ;
#7340=VERTEX_POINT ( 'NONE', #49638 ) ;
#7341=PLANE ( 'NONE',  #17309 ) ;
#7342=DIRECTION ( 'NONE',  ( 0.000000000000000000, 0.000000000000000000, 1.000000000000000000 ) ) ;
#7343=ORIENTED_EDGE ( 'NONE', *, *, #13009, .F. ) ;
#7345=FACE_OUTER_BOUND ( 'NONE', #50276, .T. ) ;
#7346=CARTESIAN_POINT ( 'NONE',  ( -5.850000000000019185, 2.500000000000000000, 6.595190528383296780 ) ) ;
#7347=DIRECTION ( 'NONE',  ( -0.000000000000000000, 1.000000000000000000, -0.000000000000000000 ) ) ;
#7349=VERTEX_POINT ( 'NONE', #121568 ) ;
#7350=CIRCLE ( 'NONE', #17822, 0.1000000000000000472 ) ;
#7351=DIRECTION ( 'NONE',  ( -0.000000000000000000, -1.000000000000000000, -0.000000000000000000 ) ) ;
#7352=PLANE ( 'NONE',  #108300 ) ;
#7354=VERTEX_POINT ( 'NONE', #111090 ) ;
#7355=AXIS2_PLACEMENT_3D ( 'NONE', #44640, #84563, #104822 ) ;
#7356=( BOUNDED_CURVE ( )  B_SPLINE_CURVE ( 2, ( #44147, #36283, #95829 ),
 .UNSPECIFIED., .F., .F. ) 
 B_SPLINE_CURVE_WITH_KNOTS ( ( 3, 3 ),
 ( -6.000000000053022403E-08, 0.01482991977946481257 ),
 .UNSPECIFIED. ) 
 CURVE ( )  GEOMETRIC_REPRESENTATION_ITEM ( )  RATIONAL_B_SPLINE_CURVE ( ( 1.000000000000000000, 0.7762344340431478473, 0.8943752373141966583 ) ) 
 REPRESENTATION_ITEM ( '' )  );
#7357=DIRECTION ( 'NONE',  ( 0.000000000000000000, 0.000000000000000000, -1.000000000000000000 ) ) ;
#7358=DIRECTION ( 'NONE',  ( 0.000000000000000000, 0.000000000000000000, -1.000000000000000000 ) ) ;
#7359=DIRECTION ( 'NONE',  ( 0.000000000000000000, 1.000000000000000000, 0.000000000000000000 ) ) ;
#7360=ADVANCED_FACE ( 'NONE', ( #29992 ), #49478, .T. ) ;
#7361=AXIS2_PLACEMENT_3D ( 'NONE', #30643, #70543, #61384 ) ;
#7362=ORIENTED_EDGE ( 'NONE', *, *, #65468, .F. ) ;
#7363=CIRCLE ( 'NONE', #78509, 0.1000000000000002554 ) ;
#7364=DIRECTION ( 'NONE',  ( -0.000000000000000000, 1.000000000000000000, -0.000000000000000000 ) ) ;
#7365=AXIS2_PLACEMENT_3D ( 'NONE', #64503, #124717, #112326 ) ;
#7366=EDGE_LOOP ( 'NONE', ( #101263, #24557, #12457, #66313 ) ) ;
#7367=LINE ( 'NONE', #86578, #60557 ) ;
#7368=DIRECTION ( 'NONE',  ( 0.000000000000000000, 0.000000000000000000, 1.000000000000000000 ) ) ;
#7369=DIRECTION ( 'NONE',  ( 0.000000000000000000, 0.000000000000000000, -1.000000000000000000 ) ) ;
#7370=ORIENTED_EDGE ( 'NONE', *, *, #107637, .F. ) ;
#7371=CIRCLE ( 'NONE', #61875, 0.09999999999999982514 ) ;
#7372=VECTOR ( 'NONE', #23696, 1000.000000000000000 ) ;
#7373=CARTESIAN_POINT ( 'NONE',  ( -5.650000000000023448, 2.500000000000000000, -6.841600689897078702 ) ) ;
#7374=CARTESIAN_POINT ( 'NONE',  ( -1.250000000000036193, 2.500000000000000000, 5.902370205355745192 ) ) ;
#7375=CONICAL_SURFACE ( 'NONE', #80566, 0.1000000000000002554, 0.003490658503988666988 ) ;
#7376=ORIENTED_EDGE ( 'NONE', *, *, #83548, .F. ) ;
#7377=DIRECTION ( 'NONE',  ( 0.000000000000000000, 0.000000000000000000, -1.000000000000000000 ) ) ;
#7378=ORIENTED_EDGE ( 'NONE', *, *, #94601, .F. ) ;
#7379=DIRECTION ( 'NONE',  ( 0.000000000000000000, -0.9999939076577903929, 0.003490651415223739937 ) ) ;
#7380=ORIENTED_EDGE ( 'NONE', *, *, #6399, .F. ) ;
#7381=CARTESIAN_POINT ( 'NONE',  ( 2.949999999999946887, 2.500000000000000000, -2.165063509461101710 ) ) ;
#7382=FACE_OUTER_BOUND ( 'NONE', #104088, .T. ) ;
#7383=EDGE_LOOP ( 'NONE', ( #108038, #7103, #97109, #30433 ) ) ;
#7384=ORIENTED_EDGE ( 'NONE', *, *, #81185, .T. ) ;
#7385=CARTESIAN_POINT ( 'NONE',  ( 8.949999999999919353, 12.50000000000000000, -6.213873640053564351 ) ) ;
#7386=CARTESIAN_POINT ( 'NONE',  ( 3.349999999999943689, 12.50000000000000000, 2.230156782645134950 ) ) ;
#7387=AXIS2_PLACEMENT_3D ( 'NONE', #122536, #32882, #53783 ) ;
#7388=ORIENTED_EDGE ( 'NONE', *, *, #120116, .F. ) ;
#7389=DIRECTION ( 'NONE',  ( 0.000000000000000000, 0.000000000000000000, 1.000000000000000000 ) ) ;
#7390=LINE ( 'NONE', #17190, #70147 ) ;
#7391=CARTESIAN_POINT ( 'NONE',  ( -3.469446951953614189E-14, 2.500000000000000000, -0.5928203230275518321 ) ) ;
#7392=CARTESIAN_POINT ( 'NONE',  ( 7.899999999999924860, 2.500000000000000000, -4.430127018922202176 ) ) ;
#7393=DIRECTION ( 'NONE',  ( -0.000000000000000000, 1.000000000000000000, -0.000000000000000000 ) ) ;
#7394=DIRECTION ( 'NONE',  ( -0.000000000000000000, 1.000000000000000000, -0.000000000000000000 ) ) ;
#7395=CIRCLE ( 'NONE', #51355, 0.06509327318403745899 ) ;
#7396=CONICAL_SURFACE ( 'NONE', #53397, 0.09999999999999999167, 0.003490658503988666988 ) ;
#7397=ADVANCED_FACE ( 'NONE', ( #60106 ), #100014, .T. ) ;
#7398=ORIENTED_EDGE ( 'NONE', *, *, #124326, .T. ) ;
#7399=ORIENTED_EDGE ( 'NONE', *, *, #20357, .F. ) ;
#7400=ORIENTED_EDGE ( 'NONE', *, *, #41893, .F. ) ;
#7401=ORIENTED_EDGE ( 'NONE', *, *, #17034, .F. ) ;
#7402=DIRECTION ( 'NONE',  ( 0.000000000000000000, 0.000000000000000000, 1.000000000000000000 ) ) ;
#7403=FACE_OUTER_BOUND ( 'NONE', #60146, .T. ) ;
#7404=CARTESIAN_POINT ( 'NONE',  ( -13.74999999999995381, 2.500000000000000000, -2.165063509461099489 ) ) ;
#7405=ORIENTED_EDGE ( 'NONE', *, *, #114862, .F. ) ;
#7406=EDGE_CURVE ( 'NONE', #64905, #26903, #15986, .T. ) ;
#7407=FACE_BOUND ( 'NONE', #92262, .T. ) ;
#7408=ADVANCED_FACE ( 'NONE', ( #1791 ), #26479, .T. ) ;
#7409=DIRECTION ( 'NONE',  ( -0.000000000000000000, 1.000000000000000000, -0.000000000000000000 ) ) ;
#7410=CARTESIAN_POINT ( 'NONE',  ( 4.349999999999940137, 12.50000000000000000, -2.576566944158915184 ) ) ;
#7412=PLANE ( 'NONE',  #95131 ) ;
#7413=DIRECTION ( 'NONE',  ( 0.000000000000000000, 1.000000000000000000, 0.000000000000000000 ) ) ;
#7414=AXIS2_PLACEMENT_3D ( 'NONE', #52820, #61366, #121549 ) ;
#7415=CARTESIAN_POINT ( 'NONE',  ( 4.349999999999940137, 12.50000000000000000, -6.841600689897078702 ) ) ;
#7416=EDGE_CURVE ( 'NONE', #32914, #58724, #10337, .T. ) ;
#7417=CARTESIAN_POINT ( 'NONE',  ( 12.49999999999993960, 12.50000000000000000, -4.265033745738164406 ) ) ;
#7418=ADVANCED_FACE ( 'NONE', ( #110468 ), #72446, .T. ) ;
#7419=PLANE ( 'NONE',  #43628 ) ;
#7420=DIRECTION ( 'NONE',  ( -0.000000000000000000, 1.000000000000000000, -0.000000000000000000 ) ) ;
#7421=ADVANCED_FACE ( 'NONE', ( #1159 ), #59470, .T. ) ;
#7422=CARTESIAN_POINT ( 'NONE',  ( 6.449999999999933564, 2.500000000000000000, -6.841600689897078702 ) ) ;
#7423=ADVANCED_FACE ( 'NONE', ( #111767 ), #53694, .T. ) ;
#7424=EDGE_CURVE ( 'NONE', #76377, #103647, #12259, .T. ) ;
#7425=DIRECTION ( 'NONE',  ( 0.000000000000000000, 0.000000000000000000, -1.000000000000000000 ) ) ;
#7426=CIRCLE ( 'NONE', #47156, 0.06509327318403745899 ) ;
#7427=ORIENTED_EDGE ( 'NONE', *, *, #3436, .T. ) ;
#7428=ORIENTED_EDGE ( 'NONE', *, *, #71201, .T. ) ;
#7429=CIRCLE ( 'NONE', #103600, 0.1000000000000000056 ) ;
#7430=ORIENTED_EDGE ( 'NONE', *, *, #108036, .T. ) ;
#7431=ORIENTED_EDGE ( 'NONE', *, *, #88462, .T. ) ;
#7432=CARTESIAN_POINT ( 'NONE',  ( -14.54999999999998472, 12.50000000000000000, 2.165063509461101265 ) ) ;
#7433=DIRECTION ( 'NONE',  ( 0.000000000000000000, 0.000000000000000000, -1.000000000000000000 ) ) ;
#7434=ORIENTED_EDGE ( 'NONE', *, *, #123458, .F. ) ;
#7435=ORIENTED_EDGE ( 'NONE', *, *, #76613, .T. ) ;
#7436=EDGE_CURVE ( 'NONE', #114403, #19267, #5648, .T. ) ;
#7437=EDGE_LOOP ( 'NONE', ( #57736, #483, #3373, #47186 ) ) ;
#7438=PLANE ( 'NONE',  #98101 ) ;
#7439=CIRCLE ( 'NONE', #67989, 0.1000000000000002554 ) ;
#7440=DIRECTION ( 'NONE',  ( 0.000000000000000000, 0.000000000000000000, 1.000000000000000000 ) ) ;
#7441=DIRECTION ( 'NONE',  ( 0.000000000000000000, 0.000000000000000000, -1.000000000000000000 ) ) ;
#7442=CARTESIAN_POINT ( 'NONE',  ( 4.149999999999939959, 2.500000000000000000, 2.757883832488649656 ) ) ;
#7443=DIRECTION ( 'NONE',  ( -4.274815082592931898E-19, -0.9999939076577903929, -0.003490651415223739937 ) ) ;
#7444=AXIS2_PLACEMENT_3D ( 'NONE', #92146, #61427, #50301 ) ;
#7445=ORIENTED_EDGE ( 'NONE', *, *, #19886, .F. ) ;
#7446=DIRECTION ( 'NONE',  ( -0.000000000000000000, 1.000000000000000000, -0.000000000000000000 ) ) ;
#7447=EDGE_LOOP ( 'NONE', ( #18985, #108648 ) ) ;
#7449=ORIENTED_EDGE ( 'NONE', *, *, #90029, .F. ) ;
#7450=ORIENTED_EDGE ( 'NONE', *, *, #20140, .T. ) ;
#7451=AXIS2_PLACEMENT_3D ( 'NONE', #21851, #33598, #113434 ) ;
#7452=DIRECTION ( 'NONE',  ( 0.000000000000000000, 1.000000000000000000, 0.000000000000000000 ) ) ;
#7453=VERTEX_POINT ( 'NONE', #109162 ) ;
#7454=EDGE_LOOP ( 'NONE', ( #53254, #54741 ) ) ;
#7455=DIRECTION ( 'NONE',  ( 0.000000000000000000, 1.000000000000000000, 0.000000000000000000 ) ) ;
#7456=VECTOR ( 'NONE', #40677, 1000.000000000000000 ) ;
#7457=DIRECTION ( 'NONE',  ( 0.000000000000000000, 0.000000000000000000, 1.000000000000000000 ) ) ;
#7458=DIRECTION ( 'NONE',  ( 0.000000000000000000, 0.000000000000000000, 1.000000000000000000 ) ) ;
#7459=CARTESIAN_POINT ( 'NONE',  ( -12.89999999999999325, 2.500000000000000000, 0.6928203230275535862 ) ) ;
#7460=AXIS2_PLACEMENT_3D ( 'NONE', #101060, #109599, #19932 ) ;
#7461=CARTESIAN_POINT ( 'NONE',  ( -6.050000000000022027, 2.500000000000000000, -6.048780366869526581 ) ) ;
#7462=ADVANCED_FACE ( 'NONE', ( #89540 ), #55836, .T. ) ;
#7463=EDGE_LOOP ( 'NONE', ( #14561, #29056 ) ) ;
#7464=ADVANCED_FACE ( 'NONE', ( #119632 ), #69910, .T. ) ;
#7465=CARTESIAN_POINT ( 'NONE',  ( -7.100000000000017408, 2.500000000000000000, 0.7928203230275495672 ) ) ;
#7466=AXIS2_PLACEMENT_3D ( 'NONE', #46790, #48726, #88637 ) ;
#7467=AXIS2_PLACEMENT_3D ( 'NONE', #41422, #14495, #102262 ) ;
#7468=ORIENTED_EDGE ( 'NONE', *, *, #72617, .F. ) ;
#7469=DIRECTION ( 'NONE',  ( 0.000000000000000000, 1.000000000000000000, 0.000000000000000000 ) ) ;
#7470=ADVANCED_FACE ( 'NONE', ( #33842 ), #112287, .T. ) ;
#7471=CIRCLE ( 'NONE', #57660, 0.1000000000000002554 ) ;
#7472=VERTEX_POINT ( 'NONE', #83601 ) ;
#7473=DIRECTION ( 'NONE',  ( -0.000000000000000000, 1.000000000000000000, -0.000000000000000000 ) ) ;
#7474=PLANE ( 'NONE',  #96331 ) ;
#7475=CONICAL_SURFACE ( 'NONE', #26270, 0.09999999999999982514, 0.003490658503988666988 ) ;
#7476=ORIENTED_EDGE ( 'NONE', *, *, #117951, .F. ) ;
#7477=CARTESIAN_POINT ( 'NONE',  ( -0.6500000000000403233, 2.500000000000000000, 6.148780366869520009 ) ) ;
#7478=EDGE_CURVE ( 'NONE', #76479, #128465, #123503, .T. ) ;
#7479=DIRECTION ( 'NONE',  ( 0.000000000000000000, 0.000000000000000000, 1.000000000000000000 ) ) ;
#7480=VERTEX_POINT ( 'NONE', #73129 ) ;
#7481=ADVANCED_FACE ( 'NONE', ( #14186 ), #54133, .T. ) ;
#7482=EDGE_CURVE ( 'NONE', #95937, #116494, #53497, .T. ) ;
#7483=ADVANCED_FACE ( 'NONE', ( #104513 ), #65223, .T. ) ;
#7484=DIRECTION ( 'NONE',  ( 0.000000000000000000, -0.9999939076577903929, 0.003490651415223739937 ) ) ;
#7485=ORIENTED_EDGE ( 'NONE', *, *, #34689, .T. ) ;
#7486=EDGE_LOOP ( 'NONE', ( #19052, #71427 ) ) ;
#7487=FACE_OUTER_BOUND ( 'NONE', #43313, .T. ) ;
#7488=CARTESIAN_POINT ( 'NONE',  ( -5.850000000000021849, 2.500000000000000000, -5.902370205355750521 ) ) ;
#7490=CIRCLE ( 'NONE', #20114, 0.06509327318403745899 ) ;
#7491=DIRECTION ( 'NONE',  ( 0.000000000000000000, -0.9999939076577903929, 0.003490651415223739937 ) ) ;
#7492=EDGE_CURVE ( 'NONE', #103959, #30016, #43694, .T. ) ;
#7493=CARTESIAN_POINT ( 'NONE',  ( 1.249999999999952038, 2.500000000000000000, 2.857883832488649301 ) ) ;
#7494=CARTESIAN_POINT ( 'NONE',  ( 0.3999999999999563904, 12.50000000000000000, 3.702399969078682407 ) ) ;
#7495=VECTOR ( 'NONE', #1945, 1000.000000000000000 ) ;
#7496=AXIS2_PLACEMENT_3D ( 'NONE', #117322, #56498, #65677 ) ;
#7497=ORIENTED_EDGE ( 'NONE', *, *, #100245, .T. ) ;
#7498=CIRCLE ( 'NONE', #53491, 0.06509327318403741736 ) ;
#7499=DIRECTION ( 'NONE',  ( -0.000000000000000000, -1.000000000000000000, -0.000000000000000000 ) ) ;
#7500=LINE ( 'NONE', #74483, #14541 ) ;
#7501=AXIS2_PLACEMENT_3D ( 'NONE', #119134, #128981, #39317 ) ;
#7502=EDGE_LOOP ( 'NONE', ( #54775, #113387 ) ) ;
#7503=CARTESIAN_POINT ( 'NONE',  ( 10.19999999999991047, 2.500000000000000000, 4.676537180435972552 ) ) ;
#7504=DIRECTION ( 'NONE',  ( -0.000000000000000000, 1.000000000000000000, -0.000000000000000000 ) ) ;
#7505=EDGE_CURVE ( 'NONE', #114231, #73752, #30735, .T. ) ;
#7506=CARTESIAN_POINT ( 'NONE',  ( 10.39999999999991154, 12.50000000000000000, 5.022947341949748790 ) ) ;
#7507=DIRECTION ( 'NONE',  ( 0.000000000000000000, 0.000000000000000000, -1.000000000000000000 ) ) ;
#7508=PLANE ( 'NONE',  #3529 ) ;
#7509=ORIENTED_EDGE ( 'NONE', *, *, #32031, .F. ) ;
#7510=VECTOR ( 'NONE', #78560, 1000.000000000000000 ) ;
#7511=CONICAL_SURFACE ( 'NONE', #26318, 0.1000000000000000472, 0.003490658503988666988 ) ;
#7512=AXIS2_PLACEMENT_3D ( 'NONE', #13862, #83891, #53165 ) ;
#7513=DIRECTION ( 'NONE',  ( -0.000000000000000000, -1.000000000000000000, -0.000000000000000000 ) ) ;
#7514=EDGE_LOOP ( 'NONE', ( #70167, #50361 ) ) ;
#7515=DIRECTION ( 'NONE',  ( -4.274815082592931898E-19, -0.9999939076577903929, -0.003490651415223739937 ) ) ;
#7516=CIRCLE ( 'NONE', #36795, 0.1000000000000002554 ) ;
#7518=ADVANCED_FACE ( 'NONE', ( #113701 ), #129033, .T. ) ;
#7519=ORIENTED_EDGE ( 'NONE', *, *, #106482, .F. ) ;
#7520=VERTEX_POINT ( 'NONE', #2431 ) ;
#7521=DIRECTION ( 'NONE',  ( 0.000000000000000000, 1.000000000000000000, 0.000000000000000000 ) ) ;
#7522=VERTEX_POINT ( 'NONE', #44304 ) ;
#7524=LINE ( 'NONE', #59889, #123658 ) ;
#7525=CARTESIAN_POINT ( 'NONE',  ( -9.150000000000005684, 2.500000000000000000, 7.288010851410849256 ) ) ;
#7526=ORIENTED_EDGE ( 'NONE', *, *, #86363, .T. ) ;
#7527=FACE_BOUND ( 'NONE', #116477, .T. ) ;
#7528=CARTESIAN_POINT ( 'NONE',  ( 7.299999999999927880, 2.500000000000000000, -4.676537180435977881 ) ) ;
#7529=ORIENTED_EDGE ( 'NONE', *, *, #45438, .F. ) ;
#7530=LINE ( 'NONE', #27180, #94591 ) ;
#7531=ADVANCED_FACE ( 'NONE', ( #82315 ), #43333, .T. ) ;
#7532=DIRECTION ( 'NONE',  ( 0.000000000000000000, 0.000000000000000000, 1.000000000000000000 ) ) ;
#7534=AXIS2_PLACEMENT_3D ( 'NONE', #73434, #102896, #83280 ) ;
#7535=ORIENTED_EDGE ( 'NONE', *, *, #123900, .T. ) ;
#7536=CIRCLE ( 'NONE', #3349, 0.06509327318403745899 ) ;
#7537=ORIENTED_EDGE ( 'NONE', *, *, #121169, .T. ) ;
#7538=DIRECTION ( 'NONE',  ( 0.000000000000000000, -0.9999939076577903929, 0.003490651415223739937 ) ) ;
#7539=LINE ( 'NONE', #37019, #24837 ) ;
#7540=CARTESIAN_POINT ( 'NONE',  ( -6.650000000000018119, 2.500000000000000000, -7.088010851410853519 ) ) ;
#7541=FACE_BOUND ( 'NONE', #105696, .T. ) ;
#7542=ORIENTED_EDGE ( 'NONE', *, *, #28007, .T. ) ;
#7543=CARTESIAN_POINT ( 'NONE',  ( 10.19999999999991047, 12.50000000000000000, 4.741630453620009789 ) ) ;
#7544=PLANE ( 'NONE',  #39759 ) ;
#7545=ORIENTED_EDGE ( 'NONE', *, *, #96313, .F. ) ;
#7546=AXIS2_PLACEMENT_3D ( 'NONE', #37634, #77533, #118752 ) ;
#7547=AXIS2_PLACEMENT_3D ( 'NONE', #117648, #65995, #36562 ) ;
#7548=CARTESIAN_POINT ( 'NONE',  ( 4.999999999999973355, 12.50000000000000000, -4.330127018922201643 ) ) ;
#7549=FACE_OUTER_BOUND ( 'NONE', #55279, .T. ) ;
#7550=DIRECTION ( 'NONE',  ( 0.000000000000000000, 1.000000000000000000, 0.000000000000000000 ) ) ;
#7551=DIRECTION ( 'NONE',  ( 0.000000000000000000, 1.000000000000000000, 0.000000000000000000 ) ) ;
#7552=DIRECTION ( 'NONE',  ( -0.000000000000000000, 1.000000000000000000, -0.000000000000000000 ) ) ;
#7553=CONICAL_SURFACE ( 'NONE', #122502, 0.1000000000000002554, 0.003490658503988666988 ) ;
#7554=CONICAL_SURFACE ( 'NONE', #1303, 0.1000000000000002554, 0.003490658503988666988 ) ;
#7555=EDGE_CURVE ( 'NONE', #106700, #53221, #84220, .T. ) ;
#7556=EDGE_LOOP ( 'NONE', ( #30673, #67472 ) ) ;
#7557=ORIENTED_EDGE ( 'NONE', *, *, #89676, .T. ) ;
#7558=VERTEX_POINT ( 'NONE', #74421 ) ;
#7559=ORIENTED_EDGE ( 'NONE', *, *, #41169, .T. ) ;
#7560=ORIENTED_EDGE ( 'NONE', *, *, #27902, .T. ) ;
#7561=CARTESIAN_POINT ( 'NONE',  ( 9.149999999999918643, 2.500000000000000000, 2.265063509461097357 ) ) ;
#7562=DIRECTION ( 'NONE',  ( 0.000000000000000000, 0.000000000000000000, -1.000000000000000000 ) ) ;
#7563=ORIENTED_EDGE ( 'NONE', *, *, #71294, .T. ) ;
#7564=FACE_BOUND ( 'NONE', #73346, .T. ) ;
#7565=EDGE_CURVE ( 'NONE', #113013, #89246, #120590, .T. ) ;
#7566=CARTESIAN_POINT ( 'NONE',  ( -2.900000000000029221, 2.500000000000000000, -0.6928203230275541413 ) ) ;
#7567=DIRECTION ( 'NONE',  ( 0.000000000000000000, 0.000000000000000000, -1.000000000000000000 ) ) ;
#7568=EDGE_CURVE ( 'NONE', #82944, #77871, #80894, .T. ) ;
#7569=CARTESIAN_POINT ( 'NONE',  ( -9.350000000000006750, 2.500000000000000000, 1.718653347947321386 ) ) ;
#7570=ADVANCED_FACE ( 'NONE', ( #42385 ), #72495, .T. ) ;
#7571=DIRECTION ( 'NONE',  ( 0.000000000000000000, -0.000000000000000000, 1.000000000000000000 ) ) ;
#7572=ADVANCED_FACE ( 'NONE', ( #122242 ), #35156, .T. ) ;
#7573=CARTESIAN_POINT ( 'NONE',  ( 15.59999999999988951, 12.50000000000000000, -0.3464101615137783474 ) ) ;
#7574=ADVANCED_FACE ( 'NONE', ( #112415 ), #16103, .T. ) ;
#7575=CIRCLE ( 'NONE', #57772, 0.06509327318403745899 ) ;
#7576=ORIENTED_EDGE ( 'NONE', *, *, #113560, .T. ) ;
#7577=DIRECTION ( 'NONE',  ( -0.000000000000000000, -1.000000000000000000, -0.000000000000000000 ) ) ;
#7578=VERTEX_POINT ( 'NONE', #105811 ) ;
#7579=CONICAL_SURFACE ( 'NONE', #51519, 0.1000000000000002554, 0.003490658503988666988 ) ;
#7580=ORIENTED_EDGE ( 'NONE', *, *, #119425, .T. ) ;
#7581=VERTEX_POINT ( 'NONE', #37720 ) ;
#7582=FACE_OUTER_BOUND ( 'NONE', #18545, .T. ) ;
#7583=CARTESIAN_POINT ( 'NONE',  ( -7.900000000000014566, 2.500000000000000000, -4.330127018922201643 ) ) ;
#7584=AXIS2_PLACEMENT_3D ( 'NONE', #66665, #127539, #28051 ) ;
#7585=FACE_OUTER_BOUND ( 'NONE', #93493, .T. ) ;
#7586=ORIENTED_EDGE ( 'NONE', *, *, #107788, .F. ) ;
#7587=EDGE_CURVE ( 'NONE', #112225, #77376, #77624, .T. ) ;
#7588=CARTESIAN_POINT ( 'NONE',  ( 10.61495711640361073, 2.500000000000000000, -8.020491764207555718 ) ) ;
#7589=VECTOR ( 'NONE', #89520, 1000.000000000000000 ) ;
#7590=CIRCLE ( 'NONE', #13845, 0.09999999999999982514 ) ;
#7591=EDGE_CURVE ( 'NONE', #39666, #33436, #116900, .T. ) ;
#7592=DIRECTION ( 'NONE',  ( -0.000000000000000000, 1.000000000000000000, -0.000000000000000000 ) ) ;
#7593=EDGE_CURVE ( 'NONE', #88166, #6702, #56683, .T. ) ;
#7594=AXIS2_PLACEMENT_3D ( 'NONE', #121698, #52972, #12391 ) ;
#7595=DIRECTION ( 'NONE',  ( -4.274815082592931898E-19, -0.9999939076577903929, -0.003490651415223739937 ) ) ;
#7597=CARTESIAN_POINT ( 'NONE',  ( -6.850000000000013856, 12.50000000000000000, 6.841600689897072485 ) ) ;
#7598=CARTESIAN_POINT ( 'NONE',  ( 11.24999999999990585, 12.50000000000000000, 2.792790559304612064 ) ) ;
#7599=CARTESIAN_POINT ( 'NONE',  ( 1.249999999999952482, 2.500000000000000000, -5.902370205355750521 ) ) ;
#7600=ORIENTED_EDGE ( 'NONE', *, *, #101081, .F. ) ;
#7601=DIRECTION ( 'NONE',  ( -0.000000000000000000, 1.000000000000000000, -0.000000000000000000 ) ) ;
#7602=AXIS2_PLACEMENT_3D ( 'NONE', #18169, #58115, #98020 ) ;
#7603=VERTEX_POINT ( 'NONE', #108384 ) ;
#7604=AXIS2_PLACEMENT_3D ( 'NONE', #103897, #121586, #52862 ) ;
#7605=CIRCLE ( 'NONE', #28552, 0.1000000000000002554 ) ;
#7607=CARTESIAN_POINT ( 'NONE',  ( 9.549999999999915445, 2.500000000000000000, -2.065063509461102065 ) ) ;
#7608=CARTESIAN_POINT ( 'NONE',  ( -8.350000000000008527, 2.500000000000000000, 5.702370205355745014 ) ) ;
#7609=DIRECTION ( 'NONE',  ( -4.274815082592931898E-19, -0.9999939076577903929, -0.003490651415223739937 ) ) ;
#7610=ORIENTED_EDGE ( 'NONE', *, *, #41003, .T. ) ;
#7611=ORIENTED_EDGE ( 'NONE', *, *, #102433, .T. ) ;
#7613=CARTESIAN_POINT ( 'NONE',  ( -8.300000000000009592, 2.500000000000000000, 4.430127018922196847 ) ) ;
#7614=LINE ( 'NONE', #47563, #115095 ) ;
#7615=VERTEX_POINT ( 'NONE', #27891 ) ;
#7616=ORIENTED_EDGE ( 'NONE', *, *, #93050, .T. ) ;
#7617=DIRECTION ( 'NONE',  ( 0.000000000000000000, 0.000000000000000000, 1.000000000000000000 ) ) ;
#7618=VERTEX_POINT ( 'NONE', #96612 ) ;
#7619=CARTESIAN_POINT ( 'NONE',  ( 9.549999999999915445, 2.500000000000000000, 6.495190528383297135 ) ) ;
#7621=ORIENTED_EDGE ( 'NONE', *, *, #9785, .T. ) ;
#7622=DIRECTION ( 'NONE',  ( 0.000000000000000000, 0.000000000000000000, -1.000000000000000000 ) ) ;
#7623=DIRECTION ( 'NONE',  ( 0.000000000000000000, 1.000000000000000000, 0.000000000000000000 ) ) ;
#7624=LINE ( 'NONE', #76388, #48880 ) ;
#7625=EDGE_CURVE ( 'NONE', #75839, #49848, #108067, .T. ) ;
#7626=CARTESIAN_POINT ( 'NONE',  ( -15.59999999999998010, 2.500000000000000000, -0.2464101615137759549 ) ) ;
#7627=ORIENTED_EDGE ( 'NONE', *, *, #126383, .F. ) ;
#7628=EDGE_CURVE ( 'NONE', #8482, #39568, #26600, .T. ) ;
#7629=CARTESIAN_POINT ( 'NONE',  ( 9.149999999999920419, 2.500000000000000000, -5.902370205355750521 ) ) ;
#7630=CIRCLE ( 'NONE', #101733, 0.06509327318403741736 ) ;
#7631=VECTOR ( 'NONE', #92183, 1000.000000000000000 ) ;
#7632=EDGE_CURVE ( 'NONE', #110466, #93340, #124803, .T. ) ;
#7633=ORIENTED_EDGE ( 'NONE', *, *, #82253, .T. ) ;
#7634=ORIENTED_EDGE ( 'NONE', *, *, #125670, .F. ) ;
#7635=PLANE ( 'NONE',  #52064 ) ;
#7636=PLANE ( 'NONE',  #26087 ) ;
#7637=PLANE ( 'NONE',  #105522 ) ;
#7638=CARTESIAN_POINT ( 'NONE',  ( -13.54999999999999005, 2.500000000000000000, 2.611473670974877148 ) ) ;
#7639=CARTESIAN_POINT ( 'NONE',  ( -6.050000000000018474, 12.50000000000000000, 2.446380397790835826 ) ) ;
#7640=EDGE_CURVE ( 'NONE', #17235, #14780, #27239, .T. ) ;
#7641=VECTOR ( 'NONE', #9938, 1000.000000000000000 ) ;
#7642=CARTESIAN_POINT ( 'NONE',  ( 3.349999999999942801, 2.500000000000000000, 2.857883832488649301 ) ) ;
#7643=PLANE ( 'NONE',  #107351 ) ;
#7644=DIRECTION ( 'NONE',  ( -0.000000000000000000, 1.000000000000000000, -0.000000000000000000 ) ) ;
#7645=FACE_OUTER_BOUND ( 'NONE', #33920, .T. ) ;
#7646=LINE ( 'NONE', #106505, #77231 ) ;
#7647=CONICAL_SURFACE ( 'NONE', #112221, 0.1000000000000002554, 0.003490658503988666988 ) ;
#7648=VECTOR ( 'NONE', #100285, 1000.000000000000000 ) ;
#7649=CONICAL_SURFACE ( 'NONE', #59921, 0.09999999999999982514, 0.003490658503988666988 ) ;
#7650=ORIENTED_EDGE ( 'NONE', *, *, #75133, .F. ) ;
#7651=FACE_OUTER_BOUND ( 'NONE', #7016, .T. ) ;
#7652=DIRECTION ( 'NONE',  ( 0.000000000000000000, 0.000000000000000000, 1.000000000000000000 ) ) ;
#7653=CARTESIAN_POINT ( 'NONE',  ( -3.100000000000028955, 2.500000000000000000, 4.576537180435972019 ) ) ;
#7654=ADVANCED_FACE ( 'NONE', ( #76994 ), #85523, .T. ) ;
#7655=DIRECTION ( 'NONE',  ( 0.000000000000000000, -0.000000000000000000, 1.000000000000000000 ) ) ;
#7656=DIRECTION ( 'NONE',  ( 0.000000000000000000, 0.000000000000000000, -1.000000000000000000 ) ) ;
#7657=ORIENTED_EDGE ( 'NONE', *, *, #101344, .F. ) ;
#7658=CARTESIAN_POINT ( 'NONE',  ( -0.8000000000000315747, 12.50000000000000000, -0.06509327318403743123 ) ) ;
#7659=PLANE ( 'NONE',  #76344 ) ;
#7660=CARTESIAN_POINT ( 'NONE',  ( -6.650000000000019007, 12.50000000000000000, -1.472243186433550122 ) ) ;
#7661=EDGE_LOOP ( 'NONE', ( #75281, #40433 ) ) ;
#7662=ORIENTED_EDGE ( 'NONE', *, *, #59030, .F. ) ;
#7663=AXIS2_PLACEMENT_3D ( 'NONE', #107574, #17892, #89854 ) ;
#7664=EDGE_CURVE ( 'NONE', #55928, #126709, #89290, .T. ) ;
#7665=VERTEX_POINT ( 'NONE', #67141 ) ;
#7666=ORIENTED_EDGE ( 'NONE', *, *, #4953, .T. ) ;
#7667=EDGE_LOOP ( 'NONE', ( #12501, #49577, #108710, #72637 ) ) ;
#7668=DIRECTION ( 'NONE',  ( 0.000000000000000000, 1.000000000000000000, 0.000000000000000000 ) ) ;
#7669=ADVANCED_FACE ( 'NONE', ( #118208 ), #122739, .T. ) ;
#7670=CIRCLE ( 'NONE', #16073, 0.09999999999999982514 ) ;
#7671=FACE_OUTER_BOUND ( 'NONE', #1547, .T. ) ;
#7672=DIRECTION ( 'NONE',  ( 0.000000000000000000, 1.000000000000000000, 0.000000000000000000 ) ) ;
#7673=AXIS2_PLACEMENT_3D ( 'NONE', #84527, #123172, #124458 ) ;
#7674=CARTESIAN_POINT ( 'NONE',  ( 12.49999999999990408, 2.500000000000000000, 5.022947341949748790 ) ) ;
#7675=VERTEX_POINT ( 'NONE', #86810 ) ;
#7676=CONICAL_SURFACE ( 'NONE', #9838, 0.1000000000000002554, 0.003490658503988666988 ) ;
#7677=CARTESIAN_POINT ( 'NONE',  ( -12.89999999999999147, 2.500000000000000000, 5.122947341949749323 ) ) ;
#7678=EDGE_LOOP ( 'NONE', ( #114807, #27182, #2412, #43129 ) ) ;
#7679=CARTESIAN_POINT ( 'NONE',  ( 26.76314062981183639, -1.072173157152068734, -4.440523076946065295 ) ) ;
#7680=CARTESIAN_POINT ( 'NONE',  ( 5.199999999999935341, 2.500000000000000000, -0.2464101615137783419 ) ) ;
#7682=DIRECTION ( 'NONE',  ( 0.000000000000000000, 0.000000000000000000, 1.000000000000000000 ) ) ;
#7683=AXIS2_PLACEMENT_3D ( 'NONE', #108061, #18393, #58341 ) ;
#7684=EDGE_CURVE ( 'NONE', #101675, #28068, #25967, .T. ) ;
#7685=DIRECTION ( 'NONE',  ( 0.000000000000000000, 1.000000000000000000, 0.000000000000000000 ) ) ;
#7686=CONICAL_SURFACE ( 'NONE', #78734, 0.1000000000000002554, 0.003490658503988666988 ) ;
#7687=VERTEX_POINT ( 'NONE', #56049 ) ;
#7688=CIRCLE ( 'NONE', #78833, 0.06509327318403745899 ) ;
#7689=AXIS2_PLACEMENT_3D ( 'NONE', #81800, #61542, #41265 ) ;
#7690=ORIENTED_EDGE ( 'NONE', *, *, #52984, .T. ) ;
#7691=EDGE_LOOP ( 'NONE', ( #54018, #124313 ) ) ;
#7692=ORIENTED_EDGE ( 'NONE', *, *, #107796, .T. ) ;
#7693=DIRECTION ( 'NONE',  ( 0.000000000000000000, 1.000000000000000000, 0.000000000000000000 ) ) ;
#7694=LINE ( 'NONE', #27994, #45682 ) ;
#7695=EDGE_CURVE ( 'NONE', #114560, #87328, #57354, .T. ) ;
#7696=PLANE ( 'NONE',  #98447 ) ;
#7697=FACE_BOUND ( 'NONE', #18858, .T. ) ;
#7698=DIRECTION ( 'NONE',  ( 0.000000000000000000, 0.000000000000000000, -1.000000000000000000 ) ) ;
#7699=CARTESIAN_POINT ( 'NONE',  ( -0.4500000000000397571, 2.500000000000000000, -2.165063509461101710 ) ) ;
#7700=CARTESIAN_POINT ( 'NONE',  ( 0.8499999999999553468, 2.500000000000000000, -2.957883832488653830 ) ) ;
#7701=DIRECTION ( 'NONE',  ( 0.000000000000000000, 0.000000000000000000, 1.000000000000000000 ) ) ;
#7703=DIRECTION ( 'NONE',  ( -0.000000000000000000, -1.000000000000000000, -0.000000000000000000 ) ) ;
#7704=AXIS2_PLACEMENT_3D ( 'NONE', #128030, #45616, #95993 ) ;
#7705=CARTESIAN_POINT ( 'NONE',  ( -7.499999999999980460, 2.500000000000000000, -4.230127018922201998 ) ) ;
#7706=LINE ( 'NONE', #105927, #118366 ) ;
#7707=ADVANCED_FACE ( 'NONE', ( #6291 ), #38379, .T. ) ;
#7708=ORIENTED_EDGE ( 'NONE', *, *, #95264, .F. ) ;
#7709=ORIENTED_EDGE ( 'NONE', *, *, #26637, .T. ) ;
#7710=EDGE_LOOP ( 'NONE', ( #124299, #97535 ) ) ;
#7711=ORIENTED_EDGE ( 'NONE', *, *, #114273, .F. ) ;
#7712=CARTESIAN_POINT ( 'NONE',  ( -15.39999999999997904, 12.50000000000000000, -0.6277270498435144619 ) ) ;
#7713=FACE_BOUND ( 'NONE', #80345, .T. ) ;
#7714=DIRECTION ( 'NONE',  ( 0.000000000000000000, 1.000000000000000000, 0.000000000000000000 ) ) ;
#7715=EDGE_CURVE ( 'NONE', #75374, #83523, #46239, .T. ) ;
#7716=CONICAL_SURFACE ( 'NONE', #80904, 0.09999999999999999167, 0.003490658503988666988 ) ;
#7717=AXIS2_PLACEMENT_3D ( 'NONE', #22831, #100089, #31359 ) ;
#7718=EDGE_LOOP ( 'NONE', ( #64382, #57063, #46579, #48442 ) ) ;
#7719=EDGE_CURVE ( 'NONE', #50950, #119162, #99764, .T. ) ;
#7720=DIRECTION ( 'NONE',  ( 0.000000000000000000, 0.000000000000000000, 1.000000000000000000 ) ) ;
#7721=EDGE_CURVE ( 'NONE', #69080, #67022, #66299, .T. ) ;
#7722=CARTESIAN_POINT ( 'NONE',  ( 6.649999999999927525, 12.50000000000000000, 2.165063509461097713 ) ) ;
#7723=EDGE_CURVE ( 'NONE', #40625, #37050, #99672, .T. ) ;
#7724=DIRECTION ( 'NONE',  ( -0.000000000000000000, -1.000000000000000000, -0.000000000000000000 ) ) ;
#7725=EDGE_CURVE ( 'NONE', #79666, #122612, #59986, .T. ) ;
#7726=ORIENTED_EDGE ( 'NONE', *, *, #20464, .T. ) ;
#7727=DIRECTION ( 'NONE',  ( -0.000000000000000000, 1.000000000000000000, -0.000000000000000000 ) ) ;
#7728=DIRECTION ( 'NONE',  ( 0.000000000000000000, 0.000000000000000000, -1.000000000000000000 ) ) ;
#7729=AXIS2_PLACEMENT_3D ( 'NONE', #73361, #93657, #113283 ) ;
#7730=VECTOR ( 'NONE', #61465, 1000.000000000000000 ) ;
#7731=ADVANCED_FACE ( 'NONE', ( #19347 ), #49490, .T. ) ;
#7732=ORIENTED_EDGE ( 'NONE', *, *, #7715, .F. ) ;
#7733=DIRECTION ( 'NONE',  ( 0.000000000000000000, -0.9999939076577903929, 0.003490651415223739937 ) ) ;
#7734=EDGE_CURVE ( 'NONE', #87808, #123263, #74710, .T. ) ;
#7735=DIRECTION ( 'NONE',  ( 0.000000000000000000, 0.000000000000000000, 1.000000000000000000 ) ) ;
#7737=CIRCLE ( 'NONE', #43279, 0.09999999999999982514 ) ;
#7738=CONICAL_SURFACE ( 'NONE', #24480, 0.1000000000000000472, 0.003490658503988666988 ) ;
#7739=EDGE_CURVE ( 'NONE', #126164, #10889, #97689, .T. ) ;
#7740=ORIENTED_EDGE ( 'NONE', *, *, #62978, .T. ) ;
#7741=CIRCLE ( 'NONE', #43282, 0.06509327318403745899 ) ;
#7742=CARTESIAN_POINT ( 'NONE',  ( 14.39999999999989555, 2.500000000000000000, -0.2464101615137782308 ) ) ;
#7743=EDGE_CURVE ( 'NONE', #29933, #45761, #83139, .T. ) ;
#7744=CARTESIAN_POINT ( 'NONE',  ( 8.349999999999919709, 2.500000000000000000, 5.802370205355744659 ) ) ;
#7745=ORIENTED_EDGE ( 'NONE', *, *, #67387, .T. ) ;
#7746=LINE ( 'NONE', #69906, #5513 ) ;
#7747=VERTEX_POINT ( 'NONE', #118849 ) ;
#7748=ORIENTED_EDGE ( 'NONE', *, *, #55762, .F. ) ;
#7749=DIRECTION ( 'NONE',  ( 0.000000000000000000, 0.000000000000000000, 1.000000000000000000 ) ) ;
#7750=ADVANCED_FACE ( 'NONE', ( #59313 ), #91434, .T. ) ;
#7751=ORIENTED_EDGE ( 'NONE', *, *, #104056, .T. ) ;
#7752=DIRECTION ( 'NONE',  ( 0.000000000000000000, 0.000000000000000000, 1.000000000000000000 ) ) ;
#7753=FACE_BOUND ( 'NONE', #23998, .T. ) ;
#7754=EDGE_LOOP ( 'NONE', ( #70761, #97724, #60995, #84845 ) ) ;
#7756=ORIENTED_EDGE ( 'NONE', *, *, #35102, .F. ) ;
#7757=DIRECTION ( 'NONE',  ( -4.274815082592931898E-19, -0.9999939076577903929, -0.003490651415223739937 ) ) ;
#7758=CARTESIAN_POINT ( 'NONE',  ( -6.900000000000019007, 2.500000000000000000, -4.083716857408426826 ) ) ;
#7759=CARTESIAN_POINT ( 'NONE',  ( 17.49862860983209956, 2.500000000000000000, 4.081131818001135336 ) ) ;
#7760=CARTESIAN_POINT ( 'NONE',  ( 10.39999999999991509, 2.500000000000000000, 0.6928203230275494784 ) ) ;
#7762=CIRCLE ( 'NONE', #70554, 0.06509327318403745899 ) ;
#7763=AXIS2_PLACEMENT_3D ( 'NONE', #114648, #103562, #84556 ) ;
#7764=VERTEX_POINT ( 'NONE', #57121 ) ;
#7765=EDGE_LOOP ( 'NONE', ( #86108, #91422 ) ) ;
#7766=CARTESIAN_POINT ( 'NONE',  ( 4.999999999999936939, 2.500000000000000000, -3.637306695894650055 ) ) ;
#7767=CIRCLE ( 'NONE', #126917, 0.09999999999999999167 ) ;
#7768=DIRECTION ( 'NONE',  ( -0.000000000000000000, 1.000000000000000000, -0.000000000000000000 ) ) ;
#7769=DIRECTION ( 'NONE',  ( 0.000000000000000000, 1.000000000000000000, 0.000000000000000000 ) ) ;
#7770=VERTEX_POINT ( 'NONE', #17841 ) ;
#7771=EDGE_LOOP ( 'NONE', ( #62878, #118701, #54082, #59593 ) ) ;
#7772=EDGE_LOOP ( 'NONE', ( #121306, #69307 ) ) ;
#7773=DIRECTION ( 'NONE',  ( -0.000000000000000000, 1.000000000000000000, -0.000000000000000000 ) ) ;
#7774=AXIS2_PLACEMENT_3D ( 'NONE', #74244, #114171, #14652 ) ;
#7775=AXIS2_PLACEMENT_3D ( 'NONE', #3714, #71826, #44281 ) ;
#7776=CARTESIAN_POINT ( 'NONE',  ( 7.099999999999928590, 2.500000000000000000, 4.430127018922196847 ) ) ;
#7777=DIRECTION ( 'NONE',  ( 0.000000000000000000, -0.9999939076577903929, 0.003490651415223739937 ) ) ;
#7778=VECTOR ( 'NONE', #96864, 1000.000000000000000 ) ;
#7780=FACE_OUTER_BOUND ( 'NONE', #125377, .T. ) ;
#7781=PLANE ( 'NONE',  #75263 ) ;
#7782=DIRECTION ( 'NONE',  ( 0.000000000000000000, 0.000000000000000000, 1.000000000000000000 ) ) ;
#7783=CARTESIAN_POINT ( 'NONE',  ( 8.749999999999918288, 2.500000000000000000, -1.472243186433550122 ) ) ;
#7784=CARTESIAN_POINT ( 'NONE',  ( -6.850000000000013856, 2.500000000000000000, 6.841600689897072485 ) ) ;
#7785=AXIS2_PLACEMENT_3D ( 'NONE', #89559, #58816, #88921 ) ;
#7786=DIRECTION ( 'NONE',  ( -0.000000000000000000, 1.000000000000000000, -0.000000000000000000 ) ) ;
#7787=VERTEX_POINT ( 'NONE', #38812 ) ;
#7788=VERTEX_POINT ( 'NONE', #78054 ) ;
#7789=EDGE_CURVE ( 'NONE', #74230, #125138, #116466, .T. ) ;
#7790=VECTOR ( 'NONE', #127889, 1000.000000000000000 ) ;
#7791=CIRCLE ( 'NONE', #18261, 0.06509327318403745899 ) ;
#7792=ADVANCED_FACE ( 'NONE', ( #98327 ), #37074, .T. ) ;
#7793=DIRECTION ( 'NONE',  ( 0.000000000000000000, -0.000000000000000000, 1.000000000000000000 ) ) ;
#7794=VERTEX_POINT ( 'NONE', #26395 ) ;
#7795=ORIENTED_EDGE ( 'NONE', *, *, #2117, .T. ) ;
#7796=DIRECTION ( 'NONE',  ( 0.000000000000000000, 0.000000000000000000, -1.000000000000000000 ) ) ;
#7797=DIRECTION ( 'NONE',  ( -0.000000000000000000, 1.000000000000000000, -0.000000000000000000 ) ) ;
#7798=CARTESIAN_POINT ( 'NONE',  ( 2.500000000000002220, 1.761799387799148686, -9.999999999999998224 ) ) ;
#7799=EDGE_CURVE ( 'NONE', #99110, #89337, #110223, .T. ) ;
#7800=DIRECTION ( 'NONE',  ( -0.000000000000000000, 1.000000000000000000, -0.000000000000000000 ) ) ;
#7801=LINE ( 'NONE', #70437, #17261 ) ;
#7802=DIRECTION ( 'NONE',  ( -0.000000000000000000, -1.000000000000000000, -0.000000000000000000 ) ) ;
#7803=DIRECTION ( 'NONE',  ( 0.000000000000000000, -0.9999939076577903929, 0.003490651415223739937 ) ) ;
#7804=ORIENTED_EDGE ( 'NONE', *, *, #85529, .T. ) ;
#7805=DIRECTION ( 'NONE',  ( -0.000000000000000000, -1.000000000000000000, -0.000000000000000000 ) ) ;
#7806=VECTOR ( 'NONE', #28971, 1000.000000000000000 ) ;
#7807=CARTESIAN_POINT ( 'NONE',  ( -4.600000000000028066, 2.500000000000000000, -5.022947341949754119 ) ) ;
#7808=ORIENTED_EDGE ( 'NONE', *, *, #52772, .T. ) ;
#7809=VERTEX_POINT ( 'NONE', #108153 ) ;
#7810=VERTEX_POINT ( 'NONE', #76777 ) ;
#7811=ORIENTED_EDGE ( 'NONE', *, *, #5263, .F. ) ;
#7812=CARTESIAN_POINT ( 'NONE',  ( 9.149999999999916866, 2.500000000000000000, 5.802370205355744659 ) ) ;
#7813=FACE_OUTER_BOUND ( 'NONE', #107584, .T. ) ;
#7814=ORIENTED_EDGE ( 'NONE', *, *, #73509, .T. ) ;
#7815=CIRCLE ( 'NONE', #93599, 0.1000000000000002554 ) ;
#7816=DIRECTION ( 'NONE',  ( 0.000000000000000000, 1.000000000000000000, 0.000000000000000000 ) ) ;
#7817=AXIS2_PLACEMENT_3D ( 'NONE', #106836, #17143, #76108 ) ;
#7818=DIRECTION ( 'NONE',  ( 0.000000000000000000, 0.000000000000000000, 1.000000000000000000 ) ) ;
#7819=DIRECTION ( 'NONE',  ( 0.000000000000000000, 0.000000000000000000, -1.000000000000000000 ) ) ;
#7820=ORIENTED_EDGE ( 'NONE', *, *, #112991, .T. ) ;
#7821=CARTESIAN_POINT ( 'NONE',  ( 11.64999999999990798, 2.500000000000000000, 7.288010851410849256 ) ) ;
#7822=CONICAL_SURFACE ( 'NONE', #32901, 0.09999999999999982514, 0.003490658503988666988 ) ;
#7823=VECTOR ( 'NONE', #64661, 1000.000000000000000 ) ;
#7824=DIRECTION ( 'NONE',  ( 0.000000000000000000, 1.000000000000000000, 0.000000000000000000 ) ) ;
#7825=EDGE_CURVE ( 'NONE', #60531, #96053, #60067, .T. ) ;
#7826=ORIENTED_EDGE ( 'NONE', *, *, #51694, .T. ) ;
#7827=AXIS2_PLACEMENT_3D ( 'NONE', #30993, #121280, #61736 ) ;
#7828=EDGE_LOOP ( 'NONE', ( #112303, #117127, #76563, #58560 ) ) ;
#7829=VERTEX_POINT ( 'NONE', #66300 ) ;
#7830=DIRECTION ( 'NONE',  ( -0.000000000000000000, 1.000000000000000000, -0.000000000000000000 ) ) ;
#7831=EDGE_CURVE ( 'NONE', #78396, #39804, #87219, .T. ) ;
#7832=AXIS2_PLACEMENT_3D ( 'NONE', #64497, #54039, #74324 ) ;
#7833=CARTESIAN_POINT ( 'NONE',  ( -9.150000000000009237, 12.50000000000000000, -6.495190528383297135 ) ) ;
#7834=CIRCLE ( 'NONE', #22453, 0.06509327318403745899 ) ;
#7835=ADVANCED_FACE ( 'NONE', ( #87220 ), #17165, .T. ) ;
#7836=ORIENTED_EDGE ( 'NONE', *, *, #64113, .T. ) ;
#7837=FACE_OUTER_BOUND ( 'NONE', #25609, .T. ) ;
#7838=CARTESIAN_POINT ( 'NONE',  ( -5.000000000000023093, 2.500000000000000000, 5.122947341949749323 ) ) ;
#7839=FACE_OUTER_BOUND ( 'NONE', #42762, .T. ) ;
#7840=CARTESIAN_POINT ( 'NONE',  ( 6.899999999999928413, 2.500000000000000000, -4.676537180435977881 ) ) ;
#7841=ORIENTED_EDGE ( 'NONE', *, *, #104007, .F. ) ;
#7842=AXIS2_PLACEMENT_3D ( 'NONE', #49905, #19789, #101567 ) ;
#7843=DIRECTION ( 'NONE',  ( 0.000000000000000000, 1.000000000000000000, 0.000000000000000000 ) ) ;
#7844=AXIS2_PLACEMENT_3D ( 'NONE', #57198, #46095, #7440 ) ;
#7845=VERTEX_POINT ( 'NONE', #127176 ) ;
#7846=ORIENTED_EDGE ( 'NONE', *, *, #34039, .T. ) ;
#7847=FACE_OUTER_BOUND ( 'NONE', #27124, .T. ) ;
#7848=ADVANCED_FACE ( 'NONE', ( #58433 ), #77413, .T. ) ;
#7849=LINE ( 'NONE', #96225, #96125 ) ;
#7850=FACE_BOUND ( 'NONE', #70360, .T. ) ;
#7851=CIRCLE ( 'NONE', #108209, 0.1000000000000002554 ) ;
#7854=CONICAL_SURFACE ( 'NONE', #41340, 0.1000000000000000472, 0.003490658503988666988 ) ;
#7855=CARTESIAN_POINT ( 'NONE',  ( 2.499999999999983569, 2.500000000000000000, -4.330127018922201643 ) ) ;
#7856=AXIS2_PLACEMENT_3D ( 'NONE', #55339, #63869, #14103 ) ;
#7857=ORIENTED_EDGE ( 'NONE', *, *, #70093, .F. ) ;
#7858=DIRECTION ( 'NONE',  ( 0.000000000000000000, 0.000000000000000000, -1.000000000000000000 ) ) ;
#7859=CARTESIAN_POINT ( 'NONE',  ( 11.44999999999990870, 12.50000000000000000, -1.818653347947326138 ) ) ;
#7860=AXIS2_PLACEMENT_3D ( 'NONE', #123200, #53171, #62348 ) ;
#7861=DIRECTION ( 'NONE',  ( -0.000000000000000000, 1.000000000000000000, -0.000000000000000000 ) ) ;
#7862=CONICAL_SURFACE ( 'NONE', #49756, 0.09999999999999982514, 0.003490658503988666988 ) ;
#7863=FACE_OUTER_BOUND ( 'NONE', #105953, .T. ) ;
#7864=ORIENTED_EDGE ( 'NONE', *, *, #100783, .T. ) ;
#7865=CARTESIAN_POINT ( 'NONE',  ( 14.59999999999989484, 12.50000000000000000, 0.6928203230275494784 ) ) ;
#7866=VECTOR ( 'NONE', #56770, 1000.000000000000000 ) ;
#7867=CARTESIAN_POINT ( 'NONE',  ( -6.050000000000022027, 2.500000000000000000, -6.248780366869526759 ) ) ;
#7868=ORIENTED_EDGE ( 'NONE', *, *, #48861, .F. ) ;
#7869=ORIENTED_EDGE ( 'NONE', *, *, #56966, .T. ) ;
#7870=CARTESIAN_POINT ( 'NONE',  ( 5.599999999999931255, 2.500000000000000000, 4.083716857408420609 ) ) ;
#7871=AXIS2_PLACEMENT_3D ( 'NONE', #5029, #25309, #125460 ) ;
#7872=CARTESIAN_POINT ( 'NONE',  ( -11.44999999999999929, 12.50000000000000000, -1.753560074763284682 ) ) ;
#7873=FACE_BOUND ( 'NONE', #28917, .T. ) ;
#7875=ADVANCED_FACE ( 'NONE', ( #56468 ), #95640, .T. ) ;
#7876=CIRCLE ( 'NONE', #58077, 0.09999999999999999167 ) ;
#7877=VECTOR ( 'NONE', #127162, 1000.000000000000000 ) ;
#7878=EDGE_LOOP ( 'NONE', ( #119565, #32451, #13461, #49508 ) ) ;
#7879=DIRECTION ( 'NONE',  ( 0.000000000000000000, 0.000000000000000000, -1.000000000000000000 ) ) ;
#7880=ORIENTED_EDGE ( 'NONE', *, *, #71614, .T. ) ;
#7881=VERTEX_POINT ( 'NONE', #106854 ) ;
#7882=CARTESIAN_POINT ( 'NONE',  ( 17.37282530749029874, 0.4689596142739324014, -5.357821376857557105 ) ) ;
#7883=EDGE_CURVE ( 'NONE', #60096, #67339, #3609, .T. ) ;
#7885=EDGE_CURVE ( 'NONE', #68909, #45780, #78721, .T. ) ;
#7886=EDGE_LOOP ( 'NONE', ( #35639, #22532 ) ) ;
#7887=DIRECTION ( 'NONE',  ( 0.000000000000000000, -0.9999939076577903929, 0.003490651415223739937 ) ) ;
#7888=CARTESIAN_POINT ( 'NONE',  ( -14.14999999999998614, 12.50000000000000000, 1.472243186433549456 ) ) ;
#7889=EDGE_CURVE ( 'NONE', #93617, #102522, #43437, .T. ) ;
#7890=ADVANCED_FACE ( 'NONE', ( #19111 ), #39242, .T. ) ;
#7891=CARTESIAN_POINT ( 'NONE',  ( 8.349999999999919709, 12.50000000000000000, -2.165063509461101710 ) ) ;
#7892=EDGE_CURVE ( 'NONE', #53227, #2985, #60161, .T. ) ;
#7893=DIRECTION ( 'NONE',  ( 0.000000000000000000, 0.000000000000000000, -1.000000000000000000 ) ) ;
#7894=VERTEX_POINT ( 'NONE', #8017 ) ;
#7895=EDGE_CURVE ( 'NONE', #43342, #125999, #127800, .T. ) ;
#7896=DIRECTION ( 'NONE',  ( 0.000000000000000000, 0.000000000000000000, -1.000000000000000000 ) ) ;
#7897=DIRECTION ( 'NONE',  ( -0.000000000000000000, 1.000000000000000000, -0.000000000000000000 ) ) ;
#7898=LINE ( 'NONE', #129004, #67890 ) ;
#7899=VERTEX_POINT ( 'NONE', #46667 ) ;
#7900=CARTESIAN_POINT ( 'NONE',  ( -8.550000000000013145, 2.500000000000000000, 2.611473670974873151 ) ) ;
#7901=VERTEX_POINT ( 'NONE', #85924 ) ;
#7902=CARTESIAN_POINT ( 'NONE',  ( 7.099999999999925926, 2.500000000000000000, 0.6928203230275494784 ) ) ;
#7903=ADVANCED_FACE ( 'NONE', ( #86580 ), #126520, .T. ) ;
#7904=EDGE_LOOP ( 'NONE', ( #64232, #66812, #57160, #91312 ) ) ;
#7905=LINE ( 'NONE', #118506, #44866 ) ;
#7906=CARTESIAN_POINT ( 'NONE',  ( 2.899999999999944844, 2.500000000000000000, 5.022947341949748790 ) ) ;
#7907=AXIS2_PLACEMENT_3D ( 'NONE', #106151, #104215, #85217 ) ;
#7908=DIRECTION ( 'NONE',  ( 0.000000000000000000, -0.000000000000000000, 1.000000000000000000 ) ) ;
#7909=DIRECTION ( 'NONE',  ( -0.000000000000000000, 1.000000000000000000, -0.000000000000000000 ) ) ;
#7910=VERTEX_POINT ( 'NONE', #125575 ) ;
#7911=CARTESIAN_POINT ( 'NONE',  ( 1.899999999999951283, 2.500000000000000000, -3.983716857408426293 ) ) ;
#7912=CARTESIAN_POINT ( 'NONE',  ( -9.350000000000006750, 2.500000000000000000, 1.718653347947321386 ) ) ;
#7914=DIRECTION ( 'NONE',  ( 0.000000000000000000, 0.000000000000000000, -1.000000000000000000 ) ) ;
#7915=FACE_OUTER_BOUND ( 'NONE', #17874, .T. ) ;
#7916=CIRCLE ( 'NONE', #47648, 0.06509327318403745899 ) ;
#7917=ORIENTED_EDGE ( 'NONE', *, *, #4298, .F. ) ;
#7918=CONICAL_SURFACE ( 'NONE', #81105, 0.1000000000000002554, 0.003490658503988666988 ) ;
#7919=AXIS2_PLACEMENT_3D ( 'NONE', #40799, #2126, #121267 ) ;
#7920=VERTEX_POINT ( 'NONE', #26746 ) ;
#7921=PLANE ( 'NONE',  #49163 ) ;
#7922=VERTEX_POINT ( 'NONE', #45749 ) ;
#7923=CARTESIAN_POINT ( 'NONE',  ( 8.149999999999923972, 2.500000000000000000, -6.048780366869526581 ) ) ;
#7924=EDGE_LOOP ( 'NONE', ( #31434, #85745, #18389, #46290 ) ) ;
#7925=VERTEX_POINT ( 'NONE', #6422 ) ;
#7926=VERTEX_POINT ( 'NONE', #37224 ) ;
#7927=DIRECTION ( 'NONE',  ( 0.000000000000000000, 0.000000000000000000, 1.000000000000000000 ) ) ;
#7928=CONICAL_SURFACE ( 'NONE', #60189, 0.1000000000000002554, 0.003490658503988666988 ) ;
#7929=PLANE ( 'NONE',  #44298 ) ;
#7930=CARTESIAN_POINT ( 'NONE',  ( 15.59999999999988951, 12.50000000000000000, 0.4115034346978109769 ) ) ;
#7932=DIRECTION ( 'NONE',  ( 0.000000000000000000, 1.000000000000000000, 0.000000000000000000 ) ) ;
#7933=DIRECTION ( 'NONE',  ( 0.000000000000000000, -0.000000000000000000, 1.000000000000000000 ) ) ;
#7934=FACE_OUTER_BOUND ( 'NONE', #61648, .T. ) ;
#7935=AXIS2_PLACEMENT_3D ( 'NONE', #125341, #124702, #46789 ) ;
#7936=DIRECTION ( 'NONE',  ( 0.000000000000000000, 0.000000000000000000, -1.000000000000000000 ) ) ;
#7937=ORIENTED_EDGE ( 'NONE', *, *, #119189, .F. ) ;
#7938=CARTESIAN_POINT ( 'NONE',  ( -2.300000000000033573, 2.500000000000000000, 0.4464101615137735513 ) ) ;
#7939=VERTEX_POINT ( 'NONE', #46370 ) ;
#7940=VECTOR ( 'NONE', #18817, 1000.000000000000000 ) ;
#7941=ORIENTED_EDGE ( 'NONE', *, *, #90504, .F. ) ;
#7942=ORIENTED_EDGE ( 'NONE', *, *, #102735, .T. ) ;
#7943=EDGE_CURVE ( 'NONE', #67339, #114052, #45109, .T. ) ;
#7944=ORIENTED_EDGE ( 'NONE', *, *, #113565, .T. ) ;
#7945=( GEOMETRIC_REPRESENTATION_CONTEXT ( 3 ) GLOBAL_UNCERTAINTY_ASSIGNED_CONTEXT ( ( #105561 ) ) GLOBAL_UNIT_ASSIGNED_CONTEXT ( ( #92451, #81986, #121922 ) ) REPRESENTATION_CONTEXT ( 'NONE', 'WORKASPACE' ) );
#7946=DIRECTION ( 'NONE',  ( 0.000000000000000000, 0.000000000000000000, -1.000000000000000000 ) ) ;
#7947=ORIENTED_EDGE ( 'NONE', *, *, #74553, .F. ) ;
#7948=VERTEX_POINT ( 'NONE', #113845 ) ;
#7949=AXIS2_PLACEMENT_3D ( 'NONE', #111442, #30342, #91174 ) ;
#7950=AXIS2_PLACEMENT_3D ( 'NONE', #38051, #129036, #119187 ) ;
#7951=ADVANCED_FACE ( 'NONE', ( #66653 ), #89389, .T. ) ;
#7952=DIRECTION ( 'NONE',  ( 0.000000000000000000, 0.000000000000000000, 1.000000000000000000 ) ) ;
#7953=CARTESIAN_POINT ( 'NONE',  ( 5.649999999999936406, 2.500000000000000000, -6.741600689897077281 ) ) ;
#7954=CONICAL_SURFACE ( 'NONE', #122897, 0.1000000000000000472, 0.003490658503988666988 ) ;
#7955=DIRECTION ( 'NONE',  ( 0.000000000000000000, 1.000000000000000000, 0.000000000000000000 ) ) ;
#7956=FACE_OUTER_BOUND ( 'NONE', #91363, .T. ) ;
#7957=FACE_OUTER_BOUND ( 'NONE', #21278, .T. ) ;
#7958=VERTEX_POINT ( 'NONE', #54275 ) ;
#7961=ORIENTED_EDGE ( 'NONE', *, *, #125765, .T. ) ;
#7962=DIRECTION ( 'NONE',  ( -0.000000000000000000, -1.000000000000000000, -0.000000000000000000 ) ) ;
#7963=EDGE_LOOP ( 'NONE', ( #116081, #45606 ) ) ;
#7964=CARTESIAN_POINT ( 'NONE',  ( -0.4500000000000397571, 12.50000000000000000, -2.165063509461101710 ) ) ;
#7965=ORIENTED_EDGE ( 'NONE', *, *, #32189, .F. ) ;
#7966=CIRCLE ( 'NONE', #91600, 0.1000000000000000472 ) ;
#7967=VERTEX_POINT ( 'NONE', #34659 ) ;
#7968=DIRECTION ( 'NONE',  ( 0.000000000000000000, -0.9999939076577903929, 0.003490651415223739937 ) ) ;
#7969=CARTESIAN_POINT ( 'NONE',  ( -4.400000000000025224, 12.50000000000000000, -0.4115034346978157509 ) ) ;
#7970=AXIS2_PLACEMENT_3D ( 'NONE', #15178, #55133, #95063 ) ;
#7971=VECTOR ( 'NONE', #121828, 1000.000000000000000 ) ;
#7972=CARTESIAN_POINT ( 'NONE',  ( 11.44999999999990692, 2.500000000000000000, 1.818653347947321475 ) ) ;
#7973=PLANE ( 'NONE',  #34013 ) ;
#7974=DIRECTION ( 'NONE',  ( -0.000000000000000000, -1.000000000000000000, -0.000000000000000000 ) ) ;
#7975=VERTEX_POINT ( 'NONE', #74555 ) ;
#7976=CARTESIAN_POINT ( 'NONE',  ( 2.049999999999950084, 2.500000000000000000, -2.065063509461102065 ) ) ;
#7977=LINE ( 'NONE', #18452, #120439 ) ;
#7978=DIRECTION ( 'NONE',  ( -0.000000000000000000, -1.000000000000000000, -0.000000000000000000 ) ) ;
#7979=CARTESIAN_POINT ( 'NONE',  ( -1.900000000000034550, 12.50000000000000000, 4.611443907251934426 ) ) ;
#7980=DIRECTION ( 'NONE',  ( 0.000000000000000000, 0.000000000000000000, 1.000000000000000000 ) ) ;
#7981=EDGE_CURVE ( 'NONE', #11241, #13143, #86291, .T. ) ;
#7982=ORIENTED_EDGE ( 'NONE', *, *, #75871, .T. ) ;
#7983=EDGE_LOOP ( 'NONE', ( #88318, #66219, #111288, #91720 ) ) ;
#7984=DIRECTION ( 'NONE',  ( -4.274815082592931898E-19, -0.9999939076577903929, -0.003490651415223739937 ) ) ;
#7985=ORIENTED_EDGE ( 'NONE', *, *, #68365, .F. ) ;
#7986=FACE_OUTER_BOUND ( 'NONE', #46504, .T. ) ;
#7987=CARTESIAN_POINT ( 'NONE',  ( -3.750000000000027534, 2.500000000000000000, 2.957883832488649389 ) ) ;
#7988=ADVANCED_FACE ( 'NONE', ( #114474 ), #24814, .T. ) ;
#7989=VECTOR ( 'NONE', #111250, 1000.000000000000000 ) ;
#7990=CONICAL_SURFACE ( 'NONE', #81166, 0.1000000000000000472, 0.003490658503988666988 ) ;
#7991=AXIS2_PLACEMENT_3D ( 'NONE', #95335, #84863, #105799 ) ;
#7992=EDGE_CURVE ( 'NONE', #73675, #58654, #129118, .T. ) ;
#7993=VERTEX_POINT ( 'NONE', #84377 ) ;
#7995=CARTESIAN_POINT ( 'NONE',  ( -7.300000000000016698, 2.500000000000000000, -0.4464101615137783252 ) ) ;
#7996=LINE ( 'NONE', #125836, #102603 ) ;
#7997=EDGE_CURVE ( 'NONE', #24371, #60396, #56820, .T. ) ;
#7998=DIRECTION ( 'NONE',  ( 0.000000000000000000, 1.000000000000000000, 0.000000000000000000 ) ) ;
#7999=ORIENTED_EDGE ( 'NONE', *, *, #24766, .T. ) ;
#8000=VECTOR ( 'NONE', #91026, 1000.000000000000000 ) ;
#8001=CIRCLE ( 'NONE', #66588, 0.06509327318403745899 ) ;
#8002=CARTESIAN_POINT ( 'NONE',  ( 9.999999999999952038, 2.500000000000000000, -0.1000000000000022815 ) ) ;
#8003=LINE ( 'NONE', #28958, #22559 ) ;
#8004=EDGE_CURVE ( 'NONE', #98964, #89242, #26109, .T. ) ;
#8005=ORIENTED_EDGE ( 'NONE', *, *, #38630, .T. ) ;
#8006=ADVANCED_FACE ( 'NONE', ( #96757 ), #12011, .T. ) ;
#8007=CARTESIAN_POINT ( 'NONE',  ( -9.150000000000009237, 2.500000000000000000, -7.188010851410848723 ) ) ;
#8008=PLANE ( 'NONE',  #95727 ) ;
#8009=CIRCLE ( 'NONE', #83247, 0.06509327318403745899 ) ;
#8010=CARTESIAN_POINT ( 'NONE',  ( -9.200000000000009948, 12.50000000000000000, -4.330127018922197202 ) ) ;
#8011=VECTOR ( 'NONE', #1901, 1000.000000000000000 ) ;
#8012=ORIENTED_EDGE ( 'NONE', *, *, #66031, .T. ) ;
#8013=DIRECTION ( 'NONE',  ( 0.000000000000000000, 1.000000000000000000, 0.000000000000000000 ) ) ;
#8014=ORIENTED_EDGE ( 'NONE', *, *, #1251, .T. ) ;
#8015=DIRECTION ( 'NONE',  ( 0.000000000000000000, 0.000000000000000000, -1.000000000000000000 ) ) ;
#8016=DIRECTION ( 'NONE',  ( 0.000000000000000000, 0.000000000000000000, -1.000000000000000000 ) ) ;
#8017=CARTESIAN_POINT ( 'NONE',  ( 0.8499999999999553468, 12.50000000000000000, 2.230156782645134950 ) ) ;
#8018=VERTEX_POINT ( 'NONE', #47042 ) ;
#8019=CARTESIAN_POINT ( 'NONE',  ( 10.19999999999991580, 2.500000000000000000, -0.4464101615137783252 ) ) ;
#8020=FACE_OUTER_BOUND ( 'NONE', #54727, .T. ) ;
#8021=AXIS2_PLACEMENT_3D ( 'NONE', #64961, #93160, #113430 ) ;
#8022=ORIENTED_EDGE ( 'NONE', *, *, #50790, .T. ) ;
#8023=DIRECTION ( 'NONE',  ( 0.000000000000000000, 0.000000000000000000, -1.000000000000000000 ) ) ;
#8024=ORIENTED_EDGE ( 'NONE', *, *, #6841, .F. ) ;
#8025=DIRECTION ( 'NONE',  ( 0.000000000000000000, 0.000000000000000000, 1.000000000000000000 ) ) ;
#8026=CONICAL_SURFACE ( 'NONE', #116692, 0.09999999999999982514, 0.003490658503988666988 ) ;
#8027=ADVANCED_FACE ( 'NONE', ( #24171 ), #58001, .T. ) ;
#8028=ORIENTED_EDGE ( 'NONE', *, *, #50513, .F. ) ;
#8029=CARTESIAN_POINT ( 'NONE',  ( -11.44999999999999751, 2.500000000000000000, -2.411473670974874306 ) ) ;
#8030=CARTESIAN_POINT ( 'NONE',  ( 8.149999999999923972, 2.500000000000000000, 2.411473670974873862 ) ) ;
#8031=VERTEX_POINT ( 'NONE', #104646 ) ;
#8032=ORIENTED_EDGE ( 'NONE', *, *, #43403, .F. ) ;
#8033=CARTESIAN_POINT ( 'NONE',  ( 3.749999999999938716, 12.50000000000000000, 7.122917578226811486 ) ) ;
#8034=DIRECTION ( 'NONE',  ( 0.000000000000000000, 0.000000000000000000, -1.000000000000000000 ) ) ;
#8035=VECTOR ( 'NONE', #57540, 1000.000000000000000 ) ;
#8036=VERTEX_POINT ( 'NONE', #94843 ) ;
#8038=DIRECTION ( 'NONE',  ( -0.000000000000000000, -1.000000000000000000, -0.000000000000000000 ) ) ;
#8040=AXIS2_PLACEMENT_3D ( 'NONE', #121821, #11221, #51818 ) ;
#8041=DIRECTION ( 'NONE',  ( 0.000000000000000000, 0.000000000000000000, -1.000000000000000000 ) ) ;
#8042=CARTESIAN_POINT ( 'NONE',  ( 10.19999999999991047, 12.50000000000000000, 4.676537180435972552 ) ) ;
#8043=EDGE_CURVE ( 'NONE', #41325, #1525, #85170, .T. ) ;
#8044=CARTESIAN_POINT ( 'NONE',  ( 11.24999999999994316, 2.500000000000000000, -6.495190528383302464 ) ) ;
#8045=CARTESIAN_POINT ( 'NONE',  ( 0.3999999999999563904, 12.50000000000000000, 3.572213422710607489 ) ) ;
#8046=CIRCLE ( 'NONE', #29000, 0.06509327318403743123 ) ;
#8047=EDGE_CURVE ( 'NONE', #108686, #74379, #65369, .T. ) ;
#8048=EDGE_CURVE ( 'NONE', #22803, #84610, #95483, .T. ) ;
#8049=ORIENTED_EDGE ( 'NONE', *, *, #16182, .T. ) ;
#8050=ORIENTED_EDGE ( 'NONE', *, *, #11237, .T. ) ;
#8051=EDGE_CURVE ( 'NONE', #78443, #34708, #28758, .T. ) ;
#8052=ORIENTED_EDGE ( 'NONE', *, *, #94040, .F. ) ;
#8053=EDGE_LOOP ( 'NONE', ( #60486, #54273 ) ) ;
#8054=FACE_OUTER_BOUND ( 'NONE', #33823, .T. ) ;
#8055=DIRECTION ( 'NONE',  ( -0.000000000000000000, -1.000000000000000000, -0.000000000000000000 ) ) ;
#8056=DIRECTION ( 'NONE',  ( 0.000000000000000000, 0.000000000000000000, -1.000000000000000000 ) ) ;
#8057=VECTOR ( 'NONE', #33197, 1000.000000000000000 ) ;
#8058=ORIENTED_EDGE ( 'NONE', *, *, #41673, .F. ) ;
#8059=FACE_BOUND ( 'NONE', #75040, .T. ) ;
#8060=ORIENTED_EDGE ( 'NONE', *, *, #85232, .T. ) ;
#8061=DIRECTION ( 'NONE',  ( 0.000000000000000000, 0.000000000000000000, 1.000000000000000000 ) ) ;
#8062=CARTESIAN_POINT ( 'NONE',  ( 7.899999999999924860, 2.500000000000000000, -4.230127018922201998 ) ) ;
#8063=EDGE_CURVE ( 'NONE', #96874, #128968, #26686, .T. ) ;
#8064=DIRECTION ( 'NONE',  ( 0.000000000000000000, 1.000000000000000000, 0.000000000000000000 ) ) ;
#8065=VECTOR ( 'NONE', #97995, 1000.000000000000000 ) ;
#8066=EDGE_CURVE ( 'NONE', #4289, #75709, #30908, .T. ) ;
#8067=CARTESIAN_POINT ( 'NONE',  ( 5.599999999999931255, 2.500000000000000000, 3.983716857408420076 ) ) ;
#8068=CARTESIAN_POINT ( 'NONE',  ( 15.83209681635537258, -2.500000000000000000, 5.404881881984332281 ) ) ;
#8069=DIRECTION ( 'NONE',  ( 0.000000000000000000, -0.000000000000000000, 1.000000000000000000 ) ) ;
#8070=DIRECTION ( 'NONE',  ( 0.000000000000000000, 0.000000000000000000, 1.000000000000000000 ) ) ;
#8071=DIRECTION ( 'NONE',  ( 0.000000000000000000, 1.000000000000000000, 0.000000000000000000 ) ) ;
#8072=DIRECTION ( 'NONE',  ( 0.000000000000000000, 0.000000000000000000, -1.000000000000000000 ) ) ;
#8073=DIRECTION ( 'NONE',  ( 0.000000000000000000, 0.000000000000000000, -1.000000000000000000 ) ) ;
#8074=ORIENTED_EDGE ( 'NONE', *, *, #94948, .T. ) ;
#8075=EDGE_LOOP ( 'NONE', ( #101310, #102742 ) ) ;
#8076=EDGE_LOOP ( 'NONE', ( #112757, #84910, #66942, #128629 ) ) ;
#8077=VERTEX_POINT ( 'NONE', #118344 ) ;
#8078=DIRECTION ( 'NONE',  ( 0.000000000000000000, -0.000000000000000000, 1.000000000000000000 ) ) ;
#8079=AXIS2_PLACEMENT_3D ( 'NONE', #1291, #100764, #111901 ) ;
#8080=DIRECTION ( 'NONE',  ( 0.000000000000000000, -0.000000000000000000, 1.000000000000000000 ) ) ;
#8081=EDGE_LOOP ( 'NONE', ( #8058, #70587 ) ) ;
#8082=ORIENTED_EDGE ( 'NONE', *, *, #80366, .F. ) ;
#8083=ORIENTED_EDGE ( 'NONE', *, *, #110786, .T. ) ;
#8084=DIRECTION ( 'NONE',  ( 0.000000000000000000, -0.000000000000000000, 1.000000000000000000 ) ) ;
#8085=VECTOR ( 'NONE', #35374, 1000.000000000000000 ) ;
#8086=CIRCLE ( 'NONE', #129405, 0.06509327318403743123 ) ;
#8087=FACE_OUTER_BOUND ( 'NONE', #95560, .T. ) ;
#8088=VECTOR ( 'NONE', #75084, 1000.000000000000000 ) ;
#8089=DIRECTION ( 'NONE',  ( 0.000000000000000000, -0.9999939076577903929, 0.003490651415223739937 ) ) ;
#8090=DIRECTION ( 'NONE',  ( -0.000000000000000000, 1.000000000000000000, -0.000000000000000000 ) ) ;
#8091=DIRECTION ( 'NONE',  ( 0.000000000000000000, 0.000000000000000000, -1.000000000000000000 ) ) ;
#8092=DIRECTION ( 'NONE',  ( -0.000000000000000000, -1.000000000000000000, -0.000000000000000000 ) ) ;
#8093=EDGE_LOOP ( 'NONE', ( #111404, #111701, #122203, #56377 ) ) ;
#8094=AXIS2_PLACEMENT_3D ( 'NONE', #45297, #85203, #26296 ) ;
#8095=VECTOR ( 'NONE', #93445, 1000.000000000000000 ) ;
#8096=CARTESIAN_POINT ( 'NONE',  ( 3.549999999999940314, 2.500000000000000000, 6.841600689897072485 ) ) ;
#8097=ORIENTED_EDGE ( 'NONE', *, *, #95572, .T. ) ;
#8098=AXIS2_PLACEMENT_3D ( 'NONE', #124505, #6610, #125755 ) ;
#8099=ORIENTED_EDGE ( 'NONE', *, *, #73288, .T. ) ;
#8100=EDGE_LOOP ( 'NONE', ( #123635, #78273 ) ) ;
#8101=VECTOR ( 'NONE', #87271, 1000.000000000000000 ) ;
#8102=DIRECTION ( 'NONE',  ( 0.000000000000000000, 1.000000000000000000, 0.000000000000000000 ) ) ;
#8103=ORIENTED_EDGE ( 'NONE', *, *, #62044, .F. ) ;
#8104=ORIENTED_EDGE ( 'NONE', *, *, #74264, .F. ) ;
#8105=AXIS2_PLACEMENT_3D ( 'NONE', #112996, #103827, #63250 ) ;
#8106=CARTESIAN_POINT ( 'NONE',  ( -4.150000000000025224, 2.500000000000000000, -1.572243186433550211 ) ) ;
#8107=EDGE_CURVE ( 'NONE', #93340, #6835, #18202, .T. ) ;
#8108=AXIS2_PLACEMENT_3D ( 'NONE', #4568, #85730, #54985 ) ;
#8109=FACE_OUTER_BOUND ( 'NONE', #15207, .T. ) ;
#8110=CARTESIAN_POINT ( 'NONE',  ( -8.750000000000010658, 12.50000000000000000, -7.188010851410848723 ) ) ;
#8111=LINE ( 'NONE', #116773, #21127 ) ;
#8112=DIRECTION ( 'NONE',  ( 0.000000000000000000, -0.000000000000000000, 1.000000000000000000 ) ) ;
#8113=ORIENTED_EDGE ( 'NONE', *, *, #22845, .F. ) ;
#8114=DIRECTION ( 'NONE',  ( 0.000000000000000000, 1.000000000000000000, 0.000000000000000000 ) ) ;
#8115=AXIS2_PLACEMENT_3D ( 'NONE', #1785, #41750, #59464 ) ;
#8116=ORIENTED_EDGE ( 'NONE', *, *, #31590, .F. ) ;
#8117=DIRECTION ( 'NONE',  ( 0.000000000000000000, 0.000000000000000000, 1.000000000000000000 ) ) ;
#8118=VERTEX_POINT ( 'NONE', #27368 ) ;
#8119=DIRECTION ( 'NONE',  ( 0.000000000000000000, 0.000000000000000000, 1.000000000000000000 ) ) ;
#8120=CARTESIAN_POINT ( 'NONE',  ( 21.25101261094845384, -0.2446824650187628403, -4.189229355218849982 ) ) ;
#8121=CIRCLE ( 'NONE', #68756, 0.1000000000000002554 ) ;
#8122=ORIENTED_EDGE ( 'NONE', *, *, #97382, .T. ) ;
#8123=DIRECTION ( 'NONE',  ( 0.000000000000000000, -0.9999939076577903929, 0.003490651415223739937 ) ) ;
#8124=CARTESIAN_POINT ( 'NONE',  ( 8.349999999999919709, 2.500000000000000000, -2.265063509461101798 ) ) ;
#8125=ORIENTED_EDGE ( 'NONE', *, *, #61431, .T. ) ;
#8126=AXIS2_PLACEMENT_3D ( 'NONE', #25853, #54646, #86701 ) ;
#8127=CARTESIAN_POINT ( 'NONE',  ( 6.249999999999932498, 12.50000000000000000, -5.737276932171712751 ) ) ;
#8128=ORIENTED_EDGE ( 'NONE', *, *, #13503, .F. ) ;
#8129=ORIENTED_EDGE ( 'NONE', *, *, #69329, .F. ) ;
#8130=CARTESIAN_POINT ( 'NONE',  ( -11.64999999999999680, 2.500000000000000000, -6.595190528383298556 ) ) ;
#8131=CARTESIAN_POINT ( 'NONE',  ( -13.34999999999999076, 2.500000000000000000, -2.165063509461099489 ) ) ;
#8133=DIRECTION ( 'NONE',  ( -0.000000000000000000, -1.000000000000000000, -0.000000000000000000 ) ) ;
#8134=AXIS2_PLACEMENT_3D ( 'NONE', #47790, #27473, #98161 ) ;
#8135=CARTESIAN_POINT ( 'NONE',  ( 10.39999999999991154, 12.50000000000000000, 5.022947341949748790 ) ) ;
#8136=DIRECTION ( 'NONE',  ( -0.000000000000000000, 1.000000000000000000, -0.000000000000000000 ) ) ;
#8137=AXIS2_PLACEMENT_3D ( 'NONE', #32436, #50759, #40302 ) ;
#8138=VERTEX_POINT ( 'NONE', #77136 ) ;
#8139=CARTESIAN_POINT ( 'NONE',  ( 8.299999999999922551, 2.500000000000000000, -2.385244779468109755E-15 ) ) ;
#8140=CARTESIAN_POINT ( 'NONE',  ( 11.04999999999991012, 2.500000000000000000, 6.841600689897072485 ) ) ;
#8141=EDGE_CURVE ( 'NONE', #103702, #33924, #3694, .T. ) ;
#8142=ORIENTED_EDGE ( 'NONE', *, *, #128917, .F. ) ;
#8143=CIRCLE ( 'NONE', #79278, 0.1000000000000002554 ) ;
#8144=VECTOR ( 'NONE', #101120, 1000.000000000000000 ) ;
#8145=EDGE_CURVE ( 'NONE', #83259, #86941, #87586, .T. ) ;
#8146=FACE_OUTER_BOUND ( 'NONE', #8303, .T. ) ;
#8147=CARTESIAN_POINT ( 'NONE',  ( 0.3999999999999563904, 12.50000000000000000, 4.957854068765711553 ) ) ;
#8148=CARTESIAN_POINT ( 'NONE',  ( 10.79999999999991012, 2.500000000000000000, 4.430127018922196847 ) ) ;
#8149=CARTESIAN_POINT ( 'NONE',  ( 9.999999999999948486, 2.500000000000000000, 4.330127018922196314 ) ) ;
#8151=DIRECTION ( 'NONE',  ( 0.000000000000000000, 1.000000000000000000, 0.000000000000000000 ) ) ;
#8152=ORIENTED_EDGE ( 'NONE', *, *, #88891, .F. ) ;
#8153=AXIS2_PLACEMENT_3D ( 'NONE', #35197, #83645, #63996 ) ;
#8154=VECTOR ( 'NONE', #73687, 1000.000000000000000 ) ;
#8155=FACE_OUTER_BOUND ( 'NONE', #58815, .T. ) ;
#8156=DIRECTION ( 'NONE',  ( 0.000000000000000000, 1.000000000000000000, 0.000000000000000000 ) ) ;
#8157=ADVANCED_FACE ( 'NONE', ( #119624 ), #58790, .T. ) ;
#8158=EDGE_CURVE ( 'NONE', #60755, #25630, #110315, .T. ) ;
#8160=ADVANCED_FACE ( 'NONE', ( #48320 ), #98058, .T. ) ;
#8161=EDGE_LOOP ( 'NONE', ( #118595, #112092 ) ) ;
#8162=CARTESIAN_POINT ( 'NONE',  ( 3.099999999999945466, 2.500000000000000000, 0.2464101615137735679 ) ) ;
#8163=ORIENTED_EDGE ( 'NONE', *, *, #35843, .F. ) ;
#8164=ORIENTED_EDGE ( 'NONE', *, *, #95668, .F. ) ;
#8165=DIRECTION ( 'NONE',  ( 0.000000000000000000, 0.000000000000000000, 1.000000000000000000 ) ) ;
#8166=AXIS2_PLACEMENT_3D ( 'NONE', #115751, #26102, #78440 ) ;
#8167=EDGE_LOOP ( 'NONE', ( #57481, #50678 ) ) ;
#8169=DIRECTION ( 'NONE',  ( -0.000000000000000000, 1.000000000000000000, -0.000000000000000000 ) ) ;
#8170=CARTESIAN_POINT ( 'NONE',  ( -6.650000000000015454, 12.50000000000000000, 7.188010851410848723 ) ) ;
#8171=ORIENTED_EDGE ( 'NONE', *, *, #39690, .T. ) ;
#8173=CARTESIAN_POINT ( 'NONE',  ( 10.64999999999991331, 2.500000000000000000, -1.918653347947325782 ) ) ;
#8174=AXIS2_PLACEMENT_3D ( 'NONE', #51621, #10390, #69969 ) ;
#8175=DIRECTION ( 'NONE',  ( -0.000000000000000000, 1.000000000000000000, -0.000000000000000000 ) ) ;
#8176=EDGE_LOOP ( 'NONE', ( #72264, #68849 ) ) ;
#8178=CARTESIAN_POINT ( 'NONE',  ( 7.699999999999922018, 12.50000000000000000, 0.3464101615137735735 ) ) ;
#8179=CONICAL_SURFACE ( 'NONE', #14432, 0.1000000000000002554, 0.003490658503988666988 ) ;
#8180=ORIENTED_EDGE ( 'NONE', *, *, #1074, .F. ) ;
#8181=CIRCLE ( 'NONE', #106488, 0.1000000000000002554 ) ;
#8182=CIRCLE ( 'NONE', #127337, 0.09999999999999982514 ) ;
#8183=EDGE_LOOP ( 'NONE', ( #66123, #22818, #23073, #113032 ) ) ;
#8184=EDGE_LOOP ( 'NONE', ( #92947, #50308 ) ) ;
#8185=FACE_OUTER_BOUND ( 'NONE', #112716, .T. ) ;
#8186=DIRECTION ( 'NONE',  ( 0.000000000000000000, 0.000000000000000000, 1.000000000000000000 ) ) ;
#8187=DIRECTION ( 'NONE',  ( 0.000000000000000000, 0.000000000000000000, 1.000000000000000000 ) ) ;
#8188=EDGE_CURVE ( 'NONE', #59250, #125502, #67270, .T. ) ;
#8189=FACE_BOUND ( 'NONE', #90233, .T. ) ;
#8190=ORIENTED_EDGE ( 'NONE', *, *, #92889, .F. ) ;
#8191=AXIS2_PLACEMENT_3D ( 'NONE', #93849, #104312, #104933 ) ;
#8192=DIRECTION ( 'NONE',  ( -0.000000000000000000, 1.000000000000000000, -0.000000000000000000 ) ) ;
#8193=CARTESIAN_POINT ( 'NONE',  ( -3.749999999999991118, 12.50000000000000000, -2.165063509461101710 ) ) ;
#8194=ORIENTED_EDGE ( 'NONE', *, *, #124342, .T. ) ;
#8195=AXIS2_PLACEMENT_3D ( 'NONE', #83027, #41182, #120368 ) ;
#8197=DIRECTION ( 'NONE',  ( 0.000000000000000000, -0.000000000000000000, 1.000000000000000000 ) ) ;
#8198=EDGE_CURVE ( 'NONE', #28988, #67778, #72757, .T. ) ;
#8199=CARTESIAN_POINT ( 'NONE',  ( -5.200000000000025935, 2.500000000000000000, -3.983716857408426293 ) ) ;
#8200=EDGE_CURVE ( 'NONE', #12706, #69185, #43535, .T. ) ;
#8201=FACE_OUTER_BOUND ( 'NONE', #108824, .T. ) ;
#8202=DIRECTION ( 'NONE',  ( -4.274815082592931898E-19, -0.9999939076577903929, -0.003490651415223739937 ) ) ;
#8203=EDGE_CURVE ( 'NONE', #11332, #36386, #95744, .T. ) ;
#8204=ORIENTED_EDGE ( 'NONE', *, *, #121688, .F. ) ;
#8205=EDGE_LOOP ( 'NONE', ( #22487, #79167, #42391, #31033 ) ) ;
#8206=EDGE_LOOP ( 'NONE', ( #88608, #23893, #872, #8050 ) ) ;
#8207=ORIENTED_EDGE ( 'NONE', *, *, #17664, .T. ) ;
#8208=EDGE_LOOP ( 'NONE', ( #115295, #1477, #129275, #55833 ) ) ;
#8209=CARTESIAN_POINT ( 'NONE',  ( -0.2000000000000412836, 12.50000000000000000, 4.741630453620009789 ) ) ;
#8210=ADVANCED_FACE ( 'NONE', ( #79085 ), #79032, .T. ) ;
#8211=DIRECTION ( 'NONE',  ( -0.000000000000000000, -1.000000000000000000, -0.000000000000000000 ) ) ;
#8212=EDGE_LOOP ( 'NONE', ( #97842, #123261, #110199, #95599 ) ) ;
#8213=EDGE_CURVE ( 'NONE', #87323, #88035, #81083, .T. ) ;
#8214=FACE_BOUND ( 'NONE', #127139, .T. ) ;
#8215=DIRECTION ( 'NONE',  ( 0.000000000000000000, 0.000000000000000000, 1.000000000000000000 ) ) ;
#8216=EDGE_CURVE ( 'NONE', #25321, #42231, #1642, .T. ) ;
#8217=ADVANCED_FACE ( 'NONE', ( #67950 ), #38526, .T. ) ;
#8219=CARTESIAN_POINT ( 'NONE',  ( -15.39999999999997904, 2.500000000000000000, 0.1000000000000000056 ) ) ;
#8220=DIRECTION ( 'NONE',  ( 0.000000000000000000, -0.000000000000000000, 1.000000000000000000 ) ) ;
#8221=CARTESIAN_POINT ( 'NONE',  ( 3.949999999999938893, 2.500000000000000000, 6.148780366869520009 ) ) ;
#8222=DIRECTION ( 'NONE',  ( 0.000000000000000000, 0.000000000000000000, 1.000000000000000000 ) ) ;
#8223=ORIENTED_EDGE ( 'NONE', *, *, #44518, .F. ) ;
#8224=AXIS2_PLACEMENT_3D ( 'NONE', #95708, #47258, #26326 ) ;
#8225=CARTESIAN_POINT ( 'NONE',  ( 17.46754094667539903, -1.506946019336847575, 5.249106724335615759 ) ) ;
#8226=EDGE_CURVE ( 'NONE', #60337, #124886, #11611, .T. ) ;
#8227=ORIENTED_EDGE ( 'NONE', *, *, #18375, .T. ) ;
#8228=ORIENTED_EDGE ( 'NONE', *, *, #104525, .T. ) ;
#8229=VERTEX_POINT ( 'NONE', #103223 ) ;
#8230=DIRECTION ( 'NONE',  ( -4.274815082592931898E-19, -0.9999939076577903929, -0.003490651415223739937 ) ) ;
#8231=CARTESIAN_POINT ( 'NONE',  ( -4.600000000000024514, 2.500000000000000000, -0.6928203230275542523 ) ) ;
#8232=DIRECTION ( 'NONE',  ( -0.000000000000000000, -1.000000000000000000, -0.000000000000000000 ) ) ;
#8233=VERTEX_POINT ( 'NONE', #1779 ) ;
#8234=LINE ( 'NONE', #39667, #22587 ) ;
#8235=DIRECTION ( 'NONE',  ( 0.000000000000000000, 1.000000000000000000, 0.000000000000000000 ) ) ;
#8236=CONICAL_SURFACE ( 'NONE', #91876, 0.1000000000000002554, 0.003490658503988666988 ) ;
#8237=DIRECTION ( 'NONE',  ( 0.000000000000000000, 0.000000000000000000, 1.000000000000000000 ) ) ;
#8238=VECTOR ( 'NONE', #111043, 1000.000000000000000 ) ;
#8239=FACE_OUTER_BOUND ( 'NONE', #55589, .T. ) ;
#8240=CARTESIAN_POINT ( 'NONE',  ( 15.79999999999989058, 12.50000000000000000, -2.385244779468109755E-15 ) ) ;
#8241=DIRECTION ( 'NONE',  ( 0.000000000000000000, 1.000000000000000000, 0.000000000000000000 ) ) ;
#8242=AXIS2_PLACEMENT_3D ( 'NONE', #80692, #40117, #70864 ) ;
#8243=DIRECTION ( 'NONE',  ( -0.000000000000000000, 1.000000000000000000, -0.000000000000000000 ) ) ;
#8244=ORIENTED_EDGE ( 'NONE', *, *, #90504, .T. ) ;
#8245=DIRECTION ( 'NONE',  ( -0.000000000000000000, -1.000000000000000000, -0.000000000000000000 ) ) ;
#8246=AXIS2_PLACEMENT_3D ( 'NONE', #9589, #120194, #41011 ) ;
#8247=AXIS2_PLACEMENT_3D ( 'NONE', #65802, #26538, #17331 ) ;
#8248=ORIENTED_EDGE ( 'NONE', *, *, #124723, .F. ) ;
#8249=ORIENTED_EDGE ( 'NONE', *, *, #81780, .F. ) ;
#8250=FACE_OUTER_BOUND ( 'NONE', #25595, .T. ) ;
#8251=DIRECTION ( 'NONE',  ( -0.000000000000000000, 1.000000000000000000, -0.000000000000000000 ) ) ;
#8252=CARTESIAN_POINT ( 'NONE',  ( 5.649999999999934630, 2.500000000000000000, 6.841600689897072485 ) ) ;
#8254=VERTEX_POINT ( 'NONE', #33212 ) ;
#8255=DIRECTION ( 'NONE',  ( -4.274815082592931898E-19, -0.9999939076577903929, -0.003490651415223739937 ) ) ;
#8256=ADVANCED_FACE ( 'NONE', ( #62665 ), #82304, .T. ) ;
#8257=CARTESIAN_POINT ( 'NONE',  ( -1.850000000000033840, 12.50000000000000000, 6.776507416713035248 ) ) ;
#8258=CARTESIAN_POINT ( 'NONE',  ( 87.50000000000001421, 0.000000000000000000, 0.000000000000000000 ) ) ;
#8259=AXIS2_PLACEMENT_3D ( 'NONE', #63781, #103704, #14007 ) ;
#8260=ORIENTED_EDGE ( 'NONE', *, *, #57897, .T. ) ;
#8261=ORIENTED_EDGE ( 'NONE', *, *, #43099, .F. ) ;
#8262=FACE_OUTER_BOUND ( 'NONE', #126531, .T. ) ;
#8263=EDGE_LOOP ( 'NONE', ( #20523, #109086, #72410, #10810 ) ) ;
#8264=DIRECTION ( 'NONE',  ( -4.274815082592931898E-19, -0.9999939076577903929, -0.003490651415223739937 ) ) ;
#8265=CIRCLE ( 'NONE', #4139, 0.06509327318403745899 ) ;
#8266=AXIS2_PLACEMENT_3D ( 'NONE', #94110, #64647, #34570 ) ;
#8267=DIRECTION ( 'NONE',  ( 0.000000000000000000, 1.000000000000000000, 0.000000000000000000 ) ) ;
#8268=EDGE_LOOP ( 'NONE', ( #110623, #121270 ) ) ;
#8269=CARTESIAN_POINT ( 'NONE',  ( 11.24999999999990763, 12.50000000000000000, -7.253104124594891289 ) ) ;
#8270=DIRECTION ( 'NONE',  ( 0.000000000000000000, 0.000000000000000000, -1.000000000000000000 ) ) ;
#8271=DIRECTION ( 'NONE',  ( 0.000000000000000000, 0.000000000000000000, -1.000000000000000000 ) ) ;
#8272=EDGE_CURVE ( 'NONE', #52442, #19417, #85270, .T. ) ;
#8273=DIRECTION ( 'NONE',  ( 0.000000000000000000, 0.000000000000000000, 1.000000000000000000 ) ) ;
#8274=ORIENTED_EDGE ( 'NONE', *, *, #119874, .T. ) ;
#8275=AXIS2_PLACEMENT_3D ( 'NONE', #109719, #10835, #99260 ) ;
#8276=VECTOR ( 'NONE', #86497, 1000.000000000000000 ) ;
#8277=AXIS2_PLACEMENT_3D ( 'NONE', #84406, #75231, #65405 ) ;
#8278=DIRECTION ( 'NONE',  ( -4.274815082592931898E-19, -0.9999939076577903929, -0.003490651415223739937 ) ) ;
#8280=EDGE_LOOP ( 'NONE', ( #26470, #65135, #103696, #120723 ) ) ;
#8281=DIRECTION ( 'NONE',  ( 0.000000000000000000, -0.000000000000000000, 1.000000000000000000 ) ) ;
#8282=DIRECTION ( 'NONE',  ( -0.000000000000000000, 1.000000000000000000, -0.000000000000000000 ) ) ;
#8283=DIRECTION ( 'NONE',  ( -0.000000000000000000, 1.000000000000000000, -0.000000000000000000 ) ) ;
#8284=DIRECTION ( 'NONE',  ( 0.000000000000000000, 1.000000000000000000, 0.000000000000000000 ) ) ;
#8286=DIRECTION ( 'NONE',  ( 0.000000000000000000, 0.000000000000000000, 1.000000000000000000 ) ) ;
#8287=CARTESIAN_POINT ( 'NONE',  ( -9.600000000000008527, 12.50000000000000000, -5.022947341949749678 ) ) ;
#8288=CONICAL_SURFACE ( 'NONE', #104439, 0.09999999999999982514, 0.003490658503988666988 ) ;
#8289=DIRECTION ( 'NONE',  ( -0.000000000000000000, 1.000000000000000000, -0.000000000000000000 ) ) ;
#8290=LINE ( 'NONE', #48227, #72069 ) ;
#8291=CARTESIAN_POINT ( 'NONE',  ( 12.09999999999990550, 2.500000000000000000, -4.230127018922201998 ) ) ;
#8292=DIRECTION ( 'NONE',  ( 0.000000000000000000, 0.000000000000000000, -1.000000000000000000 ) ) ;
#8293=AXIS2_PLACEMENT_3D ( 'NONE', #81895, #41992, #2048 ) ;
#8294=EDGE_CURVE ( 'NONE', #43428, #95183, #106209, .T. ) ;
#8295=ORIENTED_EDGE ( 'NONE', *, *, #22020, .T. ) ;
#8296=AXIS2_PLACEMENT_3D ( 'NONE', #31610, #22451, #53191 ) ;
#8297=CARTESIAN_POINT ( 'NONE',  ( 12.29999999999990479, 2.500000000000000000, -3.883716857408426648 ) ) ;
#8298=DIRECTION ( 'NONE',  ( 0.000000000000000000, 0.000000000000000000, 1.000000000000000000 ) ) ;
#8299=PLANE ( 'NONE',  #110168 ) ;
#8300=DIRECTION ( 'NONE',  ( 0.000000000000000000, 1.000000000000000000, 0.000000000000000000 ) ) ;
#8301=DIRECTION ( 'NONE',  ( 0.000000000000000000, 1.000000000000000000, 0.000000000000000000 ) ) ;
#8302=ADVANCED_FACE ( 'NONE', ( #52188 ), #122940, .T. ) ;
#8303=EDGE_LOOP ( 'NONE', ( #61559, #77245, #24599, #38359 ) ) ;
#8304=DIRECTION ( 'NONE',  ( 0.000000000000000000, 0.000000000000000000, 1.000000000000000000 ) ) ;
#8305=DIRECTION ( 'NONE',  ( 0.000000000000000000, -0.9999939076577903929, 0.003490651415223739937 ) ) ;
#8306=CARTESIAN_POINT ( 'NONE',  ( 2.949999999999945111, 2.500000000000000000, 2.265063509461097357 ) ) ;
#8307=EDGE_LOOP ( 'NONE', ( #112891, #64953, #69843, #96364 ) ) ;
#8308=EDGE_CURVE ( 'NONE', #101949, #97882, #66486, .T. ) ;
#8309=EDGE_CURVE ( 'NONE', #52226, #108554, #70531, .T. ) ;
#8310=EDGE_CURVE ( 'NONE', #81253, #64554, #83230, .T. ) ;
#8311=ADVANCED_FACE ( 'NONE', ( #52828 ), #92767, .T. ) ;
#8312=EDGE_CURVE ( 'NONE', #121486, #89530, #53981, .T. ) ;
#8313=EDGE_LOOP ( 'NONE', ( #105959, #45330 ) ) ;
#8314=CARTESIAN_POINT ( 'NONE',  ( -3.350000000000028955, 2.500000000000000000, 7.088010851410848190 ) ) ;
#8315=VERTEX_POINT ( 'NONE', #42374 ) ;
#8316=EDGE_LOOP ( 'NONE', ( #85206, #62823 ) ) ;
#8317=EDGE_LOOP ( 'NONE', ( #121951, #45089 ) ) ;
#8318=DIRECTION ( 'NONE',  ( -0.000000000000000000, 1.000000000000000000, -0.000000000000000000 ) ) ;
#8319=AXIS2_PLACEMENT_3D ( 'NONE', #76528, #124979, #75226 ) ;
#8320=EDGE_CURVE ( 'NONE', #38693, #95740, #110401, .T. ) ;
#8321=DIRECTION ( 'NONE',  ( -0.000000000000000000, -1.000000000000000000, -0.000000000000000000 ) ) ;
#8322=LINE ( 'NONE', #69168, #16939 ) ;
#8323=ADVANCED_FACE ( 'NONE', ( #61371 ), #90821, .T. ) ;
#8324=DIRECTION ( 'NONE',  ( -4.274815082592931898E-19, -0.9999939076577903929, -0.003490651415223739937 ) ) ;
#8325=EDGE_CURVE ( 'NONE', #103611, #81046, #99950, .T. ) ;
#8326=ORIENTED_EDGE ( 'NONE', *, *, #98644, .T. ) ;
#8327=CIRCLE ( 'NONE', #123267, 0.06509327318403745899 ) ;
#8328=AXIS2_PLACEMENT_3D ( 'NONE', #11422, #1591, #30445 ) ;
#8329=CARTESIAN_POINT ( 'NONE',  ( -10.60000000000000320, 2.500000000000000000, -3.983716857408421852 ) ) ;
#8330=VERTEX_POINT ( 'NONE', #41103 ) ;
#8331=DIRECTION ( 'NONE',  ( 0.000000000000000000, 0.000000000000000000, -1.000000000000000000 ) ) ;
#8332=CARTESIAN_POINT ( 'NONE',  ( 15.50772381900100605, -2.500000000000000444, -6.996973298636910421 ) ) ;
#8333=CARTESIAN_POINT ( 'NONE',  ( 21.23528140090950700, 2.699413673072311504, 2.293764360948888914 ) ) ;
#8334=FACE_OUTER_BOUND ( 'NONE', #98945, .T. ) ;
#8335=DIRECTION ( 'NONE',  ( 0.000000000000000000, -0.9999939076577903929, 0.003490651415223739937 ) ) ;
#8336=VERTEX_POINT ( 'NONE', #10940 ) ;
#8337=AXIS2_PLACEMENT_3D ( 'NONE', #124553, #93802, #74160 ) ;
#8338=AXIS2_PLACEMENT_3D ( 'NONE', #53743, #5907, #93671 ) ;
#8339=VERTEX_POINT ( 'NONE', #23351 ) ;
#8340=VERTEX_POINT ( 'NONE', #120290 ) ;
#8341=ORIENTED_EDGE ( 'NONE', *, *, #59366, .F. ) ;
#8342=VERTEX_POINT ( 'NONE', #30631 ) ;
#8343=LINE ( 'NONE', #118304, #108904 ) ;
#8344=CARTESIAN_POINT ( 'NONE',  ( -3.150000000000030553, 12.50000000000000000, 6.148780366869520009 ) ) ;
#8345=DIRECTION ( 'NONE',  ( -0.000000000000000000, 1.000000000000000000, -0.000000000000000000 ) ) ;
#8346=FACE_BOUND ( 'NONE', #28529, .T. ) ;
#8347=PLANE ( 'NONE',  #22211 ) ;
#8348=CARTESIAN_POINT ( 'NONE',  ( 0.8499999999999557909, 2.500000000000000000, -6.595190528383302109 ) ) ;
#8349=DIRECTION ( 'NONE',  ( 0.000000000000000000, -0.000000000000000000, 1.000000000000000000 ) ) ;
#8350=LINE ( 'NONE', #101900, #39672 ) ;
#8352=PLANE ( 'NONE',  #76107 ) ;
#8353=CARTESIAN_POINT ( 'NONE',  ( 9.799999999999915445, 2.500000000000000000, 3.883716857408421319 ) ) ;
#8354=AXIS2_PLACEMENT_3D ( 'NONE', #101490, #11805, #79281 ) ;
#8355=AXIS2_PLACEMENT_3D ( 'NONE', #4840, #104351, #64420 ) ;
#8356=DIRECTION ( 'NONE',  ( -0.000000000000000000, -1.000000000000000000, -0.000000000000000000 ) ) ;
#8357=EDGE_LOOP ( 'NONE', ( #16666, #25741, #103613, #79520 ) ) ;
#8358=ORIENTED_EDGE ( 'NONE', *, *, #48435, .F. ) ;
#8360=ORIENTED_EDGE ( 'NONE', *, *, #69936, .F. ) ;
#8361=FACE_OUTER_BOUND ( 'NONE', #109469, .T. ) ;
#8362=EDGE_CURVE ( 'NONE', #5223, #118122, #51835, .T. ) ;
#8363=FACE_BOUND ( 'NONE', #116783, .T. ) ;
#8364=DIRECTION ( 'NONE',  ( 0.000000000000000000, 0.000000000000000000, -1.000000000000000000 ) ) ;
#8365=EDGE_CURVE ( 'NONE', #72840, #62761, #71176, .T. ) ;
#8366=EDGE_CURVE ( 'NONE', #23090, #16470, #127147, .T. ) ;
#8367=ORIENTED_EDGE ( 'NONE', *, *, #23260, .T. ) ;
#8368=DIRECTION ( 'NONE',  ( -0.000000000000000000, -1.000000000000000000, -0.000000000000000000 ) ) ;
#8370=CARTESIAN_POINT ( 'NONE',  ( 10.64999999999990976, 2.500000000000000000, -6.841600689897077814 ) ) ;
#8371=CARTESIAN_POINT ( 'NONE',  ( 0.6499999999999561684, 2.500000000000000000, 2.611473670974873151 ) ) ;
#8372=CIRCLE ( 'NONE', #102479, 0.06509327318403745899 ) ;
#8373=ORIENTED_EDGE ( 'NONE', *, *, #31174, .T. ) ;
#8374=CARTESIAN_POINT ( 'NONE',  ( 16.55874544816229132, -0.4845305829427751232, 6.091953208798936537 ) ) ;
#8375=DIRECTION ( 'NONE',  ( 0.000000000000000000, 0.000000000000000000, -1.000000000000000000 ) ) ;
#8376=EDGE_CURVE ( 'NONE', #42757, #107800, #114955, .T. ) ;
#8377=CIRCLE ( 'NONE', #52221, 0.1000000000000002554 ) ;
#8379=ORIENTED_EDGE ( 'NONE', *, *, #4257, .T. ) ;
#8380=ORIENTED_EDGE ( 'NONE', *, *, #112845, .T. ) ;
#8381=CARTESIAN_POINT ( 'NONE',  ( -2.900000000000029665, 12.50000000000000000, 3.572213422710607489 ) ) ;
#8382=CARTESIAN_POINT ( 'NONE',  ( -12.89999999999999147, 12.50000000000000000, -0.6928203230275500335 ) ) ;
#8383=AXIS2_PLACEMENT_3D ( 'NONE', #114579, #24928, #64838 ) ;
#8384=FACE_OUTER_BOUND ( 'NONE', #67960, .T. ) ;
#8385=DIRECTION ( 'NONE',  ( 0.000000000000000000, 0.000000000000000000, -1.000000000000000000 ) ) ;
#8387=DIRECTION ( 'NONE',  ( -0.000000000000000000, 1.000000000000000000, -0.000000000000000000 ) ) ;
#8388=EDGE_LOOP ( 'NONE', ( #95082, #27655, #121407, #89385 ) ) ;
#8389=ORIENTED_EDGE ( 'NONE', *, *, #12472, .T. ) ;
#8390=DIRECTION ( 'NONE',  ( 0.000000000000000000, -0.000000000000000000, 1.000000000000000000 ) ) ;
#8392=ORIENTED_EDGE ( 'NONE', *, *, #3207, .T. ) ;
#8393=FACE_OUTER_BOUND ( 'NONE', #22035, .T. ) ;
#8394=FACE_BOUND ( 'NONE', #80469, .T. ) ;
#8395=ORIENTED_EDGE ( 'NONE', *, *, #79469, .T. ) ;
#8397=VERTEX_POINT ( 'NONE', #5004 ) ;
#8398=DIRECTION ( 'NONE',  ( 0.000000000000000000, 1.000000000000000000, 0.000000000000000000 ) ) ;
#8399=CARTESIAN_POINT ( 'NONE',  ( 8.149999999999920419, 2.500000000000000000, 6.841600689897072485 ) ) ;
#8400=DIRECTION ( 'NONE',  ( 0.000000000000000000, -0.000000000000000000, 1.000000000000000000 ) ) ;
#8401=CARTESIAN_POINT ( 'NONE',  ( 1.899999999999949507, 2.500000000000000000, 4.576537180435972019 ) ) ;
#8402=DIRECTION ( 'NONE',  ( 0.000000000000000000, 1.000000000000000000, 0.000000000000000000 ) ) ;
#8403=ORIENTED_EDGE ( 'NONE', *, *, #41940, .T. ) ;
#8405=EDGE_LOOP ( 'NONE', ( #84692, #36281 ) ) ;
#8406=DIRECTION ( 'NONE',  ( 0.000000000000000000, 0.000000000000000000, -1.000000000000000000 ) ) ;
#8407=ADVANCED_FACE ( 'NONE', ( #54747 ), #25955, .T. ) ;
#8408=DIRECTION ( 'NONE',  ( -4.274815082592931898E-19, -0.9999939076577903929, -0.003490651415223739937 ) ) ;
#8409=AXIS2_PLACEMENT_3D ( 'NONE', #97939, #88772, #77645 ) ;
#8410=DIRECTION ( 'NONE',  ( 0.000000000000000000, 0.000000000000000000, -1.000000000000000000 ) ) ;
#8411=ORIENTED_EDGE ( 'NONE', *, *, #79012, .T. ) ;
#8412=ORIENTED_EDGE ( 'NONE', *, *, #91001, .T. ) ;
#8413=ORIENTED_EDGE ( 'NONE', *, *, #36580, .F. ) ;
#8414=AXIS2_PLACEMENT_3D ( 'NONE', #84893, #54155, #114352 ) ;
#8415=CARTESIAN_POINT ( 'NONE',  ( 7.499999999999923617, 12.50000000000000000, 0.6928203230275494784 ) ) ;
#8416=DIRECTION ( 'NONE',  ( 0.000000000000000000, 0.000000000000000000, 1.000000000000000000 ) ) ;
#8418=AXIS2_PLACEMENT_3D ( 'NONE', #123308, #23830, #122664 ) ;
#8419=DIRECTION ( 'NONE',  ( 0.000000000000000000, 0.000000000000000000, 1.000000000000000000 ) ) ;
#8420=DIRECTION ( 'NONE',  ( -0.000000000000000000, 1.000000000000000000, -0.000000000000000000 ) ) ;
#8421=CARTESIAN_POINT ( 'NONE',  ( 2.299999999999949640, 12.50000000000000000, -4.741630453620015118 ) ) ;
#8422=DIRECTION ( 'NONE',  ( 0.000000000000000000, 1.000000000000000000, 0.000000000000000000 ) ) ;
#8423=DIRECTION ( 'NONE',  ( 0.000000000000000000, 1.000000000000000000, 0.000000000000000000 ) ) ;
#8424=ADVANCED_FACE ( 'NONE', ( #14176 ), #22609, .T. ) ;
#8426=ORIENTED_EDGE ( 'NONE', *, *, #87344, .F. ) ;
#8427=EDGE_LOOP ( 'NONE', ( #87769, #7196 ) ) ;
#8428=CARTESIAN_POINT ( 'NONE',  ( -5.450000000000023270, 2.500000000000000000, -2.165063509461101710 ) ) ;
#8429=LINE ( 'NONE', #96813, #40361 ) ;
#8430=EDGE_LOOP ( 'NONE', ( #61417, #110873, #79793, #20748 ) ) ;
#8431=ORIENTED_EDGE ( 'NONE', *, *, #127741, .T. ) ;
#8433=CARTESIAN_POINT ( 'NONE',  ( -6.450000000000016165, 2.500000000000000000, 2.611473670974873151 ) ) ;
#8434=DIRECTION ( 'NONE',  ( -0.000000000000000000, 1.000000000000000000, -0.000000000000000000 ) ) ;
#8435=DIRECTION ( 'NONE',  ( 0.000000000000000000, 1.000000000000000000, 0.000000000000000000 ) ) ;
#8436=DIRECTION ( 'NONE',  ( -0.000000000000000000, 1.000000000000000000, -0.000000000000000000 ) ) ;
#8437=DIRECTION ( 'NONE',  ( 0.000000000000000000, -0.9999939076577903929, 0.003490651415223739937 ) ) ;
#8438=DIRECTION ( 'NONE',  ( -0.000000000000000000, 1.000000000000000000, -0.000000000000000000 ) ) ;
#8439=DIRECTION ( 'NONE',  ( 0.000000000000000000, 1.000000000000000000, 0.000000000000000000 ) ) ;
#8440=AXIS2_PLACEMENT_3D ( 'NONE', #14369, #45154, #62847 ) ;
#8441=AXIS2_PLACEMENT_3D ( 'NONE', #10367, #81055, #128885 ) ;
#8442=ORIENTED_EDGE ( 'NONE', *, *, #115310, .F. ) ;
#8443=EDGE_CURVE ( 'NONE', #37002, #26544, #56672, .T. ) ;
#8444=VERTEX_POINT ( 'NONE', #55414 ) ;
#8445=EDGE_LOOP ( 'NONE', ( #41303, #47119, #35176, #39534 ) ) ;
#8446=ORIENTED_EDGE ( 'NONE', *, *, #39849, .T. ) ;
#8447=DIRECTION ( 'NONE',  ( -0.000000000000000000, 1.000000000000000000, -0.000000000000000000 ) ) ;
#8448=DIRECTION ( 'NONE',  ( -0.000000000000000000, -1.000000000000000000, -0.000000000000000000 ) ) ;
#8449=CIRCLE ( 'NONE', #75356, 0.06509327318403745899 ) ;
#8450=ADVANCED_FACE ( 'NONE', ( #65868 ), #18367, .T. ) ;
#8451=ORIENTED_EDGE ( 'NONE', *, *, #93414, .F. ) ;
#8452=DIRECTION ( 'NONE',  ( -4.274815082592931898E-19, -0.9999939076577903929, -0.003490651415223739937 ) ) ;
#8453=FACE_OUTER_BOUND ( 'NONE', #27917, .T. ) ;
#8454=CARTESIAN_POINT ( 'NONE',  ( 1.649999999999951950, 12.50000000000000000, -7.253104124594891289 ) ) ;
#8455=CARTESIAN_POINT ( 'NONE',  ( -0.6000000000000323963, 2.500000000000000000, -0.2464101615137759549 ) ) ;
#8456=ORIENTED_EDGE ( 'NONE', *, *, #35563, .T. ) ;
#8457=EDGE_CURVE ( 'NONE', #117477, #115271, #46228, .T. ) ;
#8458=EDGE_CURVE ( 'NONE', #75790, #82453, #82949, .T. ) ;
#8459=ADVANCED_FACE ( 'NONE', ( #24665 ), #58098, .T. ) ;
#8460=FACE_OUTER_BOUND ( 'NONE', #85640, .T. ) ;
#8461=ADVANCED_FACE ( 'NONE', ( #3724 ), #99633, .T. ) ;
#8462=CARTESIAN_POINT ( 'NONE',  ( 9.199999999999915801, 2.500000000000000000, -4.330127018922201643 ) ) ;
#8463=VECTOR ( 'NONE', #122478, 1000.000000000000000 ) ;
#8464=ORIENTED_EDGE ( 'NONE', *, *, #129123, .F. ) ;
#8465=CIRCLE ( 'NONE', #69115, 0.06509327318403745899 ) ;
#8466=ORIENTED_EDGE ( 'NONE', *, *, #118135, .F. ) ;
#8467=EDGE_CURVE ( 'NONE', #121109, #98383, #16100, .T. ) ;
#8468=ORIENTED_EDGE ( 'NONE', *, *, #125947, .T. ) ;
#8469=CARTESIAN_POINT ( 'NONE',  ( 6.849999999999929479, 2.500000000000000000, 6.841600689897072485 ) ) ;
#8470=EDGE_CURVE ( 'NONE', #111058, #89282, #44302, .T. ) ;
#8471=EDGE_CURVE ( 'NONE', #62189, #7899, #92326, .T. ) ;
#8472=CIRCLE ( 'NONE', #2135, 0.09999999999999982514 ) ;
#8473=CARTESIAN_POINT ( 'NONE',  ( -10.80000000000000071, 2.500000000000000000, 4.430127018922196847 ) ) ;
#8474=ADVANCED_FACE ( 'NONE', ( #43679 ), #25415, .T. ) ;
#8475=EDGE_CURVE ( 'NONE', #30036, #72978, #94044, .T. ) ;
#8476=VERTEX_POINT ( 'NONE', #84211 ) ;
#8477=CARTESIAN_POINT ( 'NONE',  ( -10.60000000000000320, 2.500000000000000000, -4.676537180435973440 ) ) ;
#8478=DIRECTION ( 'NONE',  ( 0.000000000000000000, -0.9999939076577903929, 0.003490651415223739937 ) ) ;
#8479=CARTESIAN_POINT ( 'NONE',  ( -14.59999999999998366, 2.500000000000000000, -1.084202172485504434E-16 ) ) ;
#8480=CARTESIAN_POINT ( 'NONE',  ( 10.59999999999990905, 2.500000000000000000, -4.676537180435978769 ) ) ;
#8481=ADVANCED_FACE ( 'NONE', ( #34503 ), #35903, .T. ) ;
#8482=VERTEX_POINT ( 'NONE', #39026 ) ;
#8483=PLANE ( 'NONE',  #85506 ) ;
#8484=ORIENTED_EDGE ( 'NONE', *, *, #48218, .T. ) ;
#8485=EDGE_LOOP ( 'NONE', ( #127037, #97002, #22676, #33810 ) ) ;
#8486=PLANE ( 'NONE',  #106133 ) ;
#8487=DIRECTION ( 'NONE',  ( 0.000000000000000000, 1.000000000000000000, 0.000000000000000000 ) ) ;
#8488=FACE_BOUND ( 'NONE', #94727, .T. ) ;
#8489=DIRECTION ( 'NONE',  ( -4.274815082592931898E-19, -0.9999939076577903929, -0.003490651415223739937 ) ) ;
#8490=DIRECTION ( 'NONE',  ( 0.000000000000000000, 1.000000000000000000, 0.000000000000000000 ) ) ;
#8491=CARTESIAN_POINT ( 'NONE',  ( -7.499999999999980460, 12.50000000000000000, 0.06509327318403515528 ) ) ;
#8492=AXIS2_PLACEMENT_3D ( 'NONE', #34380, #63827, #125315 ) ;
#8493=AXIS2_PLACEMENT_3D ( 'NONE', #32315, #11991, #12629 ) ;
#8494=EDGE_LOOP ( 'NONE', ( #55014, #66803 ) ) ;
#8495=DIRECTION ( 'NONE',  ( 0.000000000000000000, -0.000000000000000000, 1.000000000000000000 ) ) ;
#8496=AXIS2_PLACEMENT_3D ( 'NONE', #112916, #101169, #71702 ) ;
#8497=CARTESIAN_POINT ( 'NONE',  ( -5.600000000000020073, 2.500000000000000000, 3.883716857408421319 ) ) ;
#8498=DIRECTION ( 'NONE',  ( -0.000000000000000000, -1.000000000000000000, -0.000000000000000000 ) ) ;
#8499=CARTESIAN_POINT ( 'NONE',  ( 6.249999999999930722, 12.50000000000000000, -1.472243186433550122 ) ) ;
#8500=EDGE_LOOP ( 'NONE', ( #71227, #12603 ) ) ;
#8501=DIRECTION ( 'NONE',  ( 0.000000000000000000, 0.000000000000000000, 1.000000000000000000 ) ) ;
#8502=AXIS2_PLACEMENT_3D ( 'NONE', #111338, #89143, #118600 ) ;
#8503=DIRECTION ( 'NONE',  ( -0.000000000000000000, -1.000000000000000000, -0.000000000000000000 ) ) ;
#8504=EDGE_LOOP ( 'NONE', ( #92715, #32131 ) ) ;
#8506=AXIS2_PLACEMENT_3D ( 'NONE', #67149, #107092, #17416 ) ;
#8507=FACE_OUTER_BOUND ( 'NONE', #15720, .T. ) ;
#8508=DIRECTION ( 'NONE',  ( 0.000000000000000000, 0.000000000000000000, 1.000000000000000000 ) ) ;
#8509=FACE_BOUND ( 'NONE', #49345, .T. ) ;
#8510=LINE ( 'NONE', #96903, #82840 ) ;
#8512=ORIENTED_EDGE ( 'NONE', *, *, #103601, .F. ) ;
#8514=EDGE_CURVE ( 'NONE', #93080, #40679, #63087, .T. ) ;
#8515=ORIENTED_EDGE ( 'NONE', *, *, #14249, .F. ) ;
#8516=EDGE_LOOP ( 'NONE', ( #120678, #30350, #50604, #102740 ) ) ;
#8517=DIRECTION ( 'NONE',  ( 0.000000000000000000, 1.000000000000000000, 0.000000000000000000 ) ) ;
#8519=ORIENTED_EDGE ( 'NONE', *, *, #40992, .F. ) ;
#8520=LINE ( 'NONE', #48466, #13452 ) ;
#8521=DIRECTION ( 'NONE',  ( 0.000000000000000000, 0.000000000000000000, -1.000000000000000000 ) ) ;
#8523=EDGE_CURVE ( 'NONE', #71810, #88786, #18047, .T. ) ;
#8524=CARTESIAN_POINT ( 'NONE',  ( 4.399999999999940847, 12.50000000000000000, -3.918623584224389056 ) ) ;
#8525=CARTESIAN_POINT ( 'NONE',  ( 8.149999999999923972, 2.500000000000000000, -6.941600689897077459 ) ) ;
#8526=ORIENTED_EDGE ( 'NONE', *, *, #2569, .F. ) ;
#8527=FACE_OUTER_BOUND ( 'NONE', #42387, .T. ) ;
#8528=DIRECTION ( 'NONE',  ( 0.000000000000000000, 1.000000000000000000, 0.000000000000000000 ) ) ;
#8529=DIRECTION ( 'NONE',  ( 0.000000000000000000, -0.9999939076577903929, 0.003490651415223739937 ) ) ;
#8531=ORIENTED_EDGE ( 'NONE', *, *, #49281, .F. ) ;
#8532=CARTESIAN_POINT ( 'NONE',  ( -8.350000000000013856, 2.500000000000000000, -7.088010851410848190 ) ) ;
#8533=VERTEX_POINT ( 'NONE', #119470 ) ;
#8534=CARTESIAN_POINT ( 'NONE',  ( 10.59999999999991260, 2.500000000000000000, 0.4464101615137735513 ) ) ;
#8535=AXIS2_PLACEMENT_3D ( 'NONE', #4946, #122808, #73063 ) ;
#8536=ORIENTED_EDGE ( 'NONE', *, *, #18656, .T. ) ;
#8537=DIRECTION ( 'NONE',  ( -0.000000000000000000, 1.000000000000000000, -0.000000000000000000 ) ) ;
#8538=AXIS2_PLACEMENT_3D ( 'NONE', #42600, #92979, #72052 ) ;
#8539=FACE_OUTER_BOUND ( 'NONE', #65931, .T. ) ;
#8540=DIRECTION ( 'NONE',  ( 0.000000000000000000, 0.000000000000000000, -1.000000000000000000 ) ) ;
#8541=DIRECTION ( 'NONE',  ( -4.274815082592931898E-19, -0.9999939076577903929, -0.003490651415223739937 ) ) ;
#8542=EDGE_LOOP ( 'NONE', ( #84074, #5186 ) ) ;
#8543=CARTESIAN_POINT ( 'NONE',  ( 9.149999999999920419, 2.500000000000000000, 1.472243186433545459 ) ) ;
#8544=LINE ( 'NONE', #7912, #83625 ) ;
#8545=CARTESIAN_POINT ( 'NONE',  ( -9.350000000000004974, 2.500000000000000000, 6.048780366869521252 ) ) ;
#8547=DIRECTION ( 'NONE',  ( 0.000000000000000000, 0.000000000000000000, -1.000000000000000000 ) ) ;
#8548=FACE_OUTER_BOUND ( 'NONE', #117629, .T. ) ;
#8549=CIRCLE ( 'NONE', #85916, 0.06509327318403745899 ) ;
#8550=EDGE_CURVE ( 'NONE', #76648, #112463, #119517, .T. ) ;
#8551=VERTEX_POINT ( 'NONE', #48169 ) ;
#8552=AXIS2_PLACEMENT_3D ( 'NONE', #123448, #115547, #35099 ) ;
#8553=ORIENTED_EDGE ( 'NONE', *, *, #72074, .F. ) ;
#8554=DIRECTION ( 'NONE',  ( -0.000000000000000000, -1.000000000000000000, -0.000000000000000000 ) ) ;
#8555=ORIENTED_EDGE ( 'NONE', *, *, #106937, .F. ) ;
#8556=CARTESIAN_POINT ( 'NONE',  ( -9.150000000000009237, 2.500000000000000000, 2.165063509461097713 ) ) ;
#8557=ORIENTED_EDGE ( 'NONE', *, *, #23867, .F. ) ;
#8558=ORIENTED_EDGE ( 'NONE', *, *, #35848, .F. ) ;
#8559=EDGE_LOOP ( 'NONE', ( #52526, #97411 ) ) ;
#8560=CARTESIAN_POINT ( 'NONE',  ( 12.04999999999990479, 12.50000000000000000, 2.099970236277060032 ) ) ;
#8561=CARTESIAN_POINT ( 'NONE',  ( 6.649999999999929301, 2.500000000000000000, -2.165063509461101710 ) ) ;
#8562=DIRECTION ( 'NONE',  ( -4.274815082592931898E-19, -0.9999939076577903929, -0.003490651415223739937 ) ) ;
#8564=DIRECTION ( 'NONE',  ( 0.000000000000000000, 1.000000000000000000, 0.000000000000000000 ) ) ;
#8565=VECTOR ( 'NONE', #122044, 1000.000000000000000 ) ;
#8567=ADVANCED_FACE ( 'NONE', ( #6919 ), #97901, .T. ) ;
#8568=PLANE ( 'NONE',  #91557 ) ;
#8569=DIRECTION ( 'NONE',  ( -0.000000000000000000, 1.000000000000000000, -0.000000000000000000 ) ) ;
#8570=EDGE_CURVE ( 'NONE', #114031, #5343, #65123, .T. ) ;
#8571=CARTESIAN_POINT ( 'NONE',  ( 2.299999999999949640, 12.50000000000000000, -0.4115034346978156399 ) ) ;
#8572=ORIENTED_EDGE ( 'NONE', *, *, #43928, .T. ) ;
#8573=ORIENTED_EDGE ( 'NONE', *, *, #77296, .F. ) ;
#8574=ORIENTED_EDGE ( 'NONE', *, *, #14693, .F. ) ;
#8575=CARTESIAN_POINT ( 'NONE',  ( -11.89999999999999680, 2.500000000000000000, 0.3464101615137776813 ) ) ;
#8576=ORIENTED_EDGE ( 'NONE', *, *, #26237, .T. ) ;
#8577=EDGE_CURVE ( 'NONE', #28877, #108367, #88192, .T. ) ;
#8578=ORIENTED_EDGE ( 'NONE', *, *, #82982, .T. ) ;
#8579=CARTESIAN_POINT ( 'NONE',  ( -12.29999999999999361, 12.50000000000000000, 4.048810130592458201 ) ) ;
#8580=DIRECTION ( 'NONE',  ( 0.000000000000000000, 1.000000000000000000, 0.000000000000000000 ) ) ;
#8581=CARTESIAN_POINT ( 'NONE',  ( -10.20000000000000462, 12.50000000000000000, 4.676537180435972552 ) ) ;
#8582=DIRECTION ( 'NONE',  ( 0.000000000000000000, 0.000000000000000000, 1.000000000000000000 ) ) ;
#8583=CARTESIAN_POINT ( 'NONE',  ( 13.14999999999989733, 2.500000000000000000, -2.511473670974877948 ) ) ;
#8584=AXIS2_PLACEMENT_3D ( 'NONE', #111970, #32783, #62861 ) ;
#8585=CARTESIAN_POINT ( 'NONE',  ( 0.3999999999999555023, 2.500000000000000000, 4.430127018922196847 ) ) ;
#8586=VERTEX_POINT ( 'NONE', #97263 ) ;
#8587=CONICAL_SURFACE ( 'NONE', #31605, 0.09999999999999999167, 0.003490658503988666988 ) ;
#8588=DIRECTION ( 'NONE',  ( -4.274815082592931898E-19, -0.9999939076577903929, -0.003490651415223739937 ) ) ;
#8589=VERTEX_POINT ( 'NONE', #88057 ) ;
#8590=CARTESIAN_POINT ( 'NONE',  ( 14.39999999999989555, 2.500000000000000000, 0.2464101615137736789 ) ) ;
#8591=AXIS2_PLACEMENT_3D ( 'NONE', #123120, #113945, #102811 ) ;
#8592=ORIENTED_EDGE ( 'NONE', *, *, #8047, .T. ) ;
#8593=CARTESIAN_POINT ( 'NONE',  ( -10.40000000000000213, 12.50000000000000000, -4.265033745738159965 ) ) ;
#8594=ORIENTED_EDGE ( 'NONE', *, *, #46619, .T. ) ;
#8595=AXIS2_PLACEMENT_3D ( 'NONE', #15975, #94545, #4226 ) ;
#8596=ORIENTED_EDGE ( 'NONE', *, *, #110889, .T. ) ;
#8597=CARTESIAN_POINT ( 'NONE',  ( 11.44999999999990692, 12.50000000000000000, -6.776507416713040577 ) ) ;
#8598=CARTESIAN_POINT ( 'NONE',  ( -8.150000000000009237, 12.50000000000000000, 6.148780366869520009 ) ) ;
#8599=EDGE_CURVE ( 'NONE', #113919, #18774, #99408, .T. ) ;
#8600=DIRECTION ( 'NONE',  ( -4.274815082592931898E-19, -0.9999939076577903929, -0.003490651415223739937 ) ) ;
#8601=CARTESIAN_POINT ( 'NONE',  ( -10.80000000000000071, 12.50000000000000000, -2.276824562219559311E-15 ) ) ;
#8602=LINE ( 'NONE', #78676, #93180 ) ;
#8603=VERTEX_POINT ( 'NONE', #28532 ) ;
#8604=CARTESIAN_POINT ( 'NONE',  ( 6.049999999999930544, 2.500000000000000000, 2.411473670974873862 ) ) ;
#8605=CARTESIAN_POINT ( 'NONE',  ( -2.100000000000033396, 2.500000000000000000, 0.6928203230275494784 ) ) ;
#8606=EDGE_CURVE ( 'NONE', #120306, #85725, #75592, .T. ) ;
#8607=CARTESIAN_POINT ( 'NONE',  ( -5.200000000000024158, 2.500000000000000000, -4.576537180435977348 ) ) ;
#8608=EDGE_CURVE ( 'NONE', #38064, #55936, #125762, .T. ) ;
#8609=LINE ( 'NONE', #129084, #34762 ) ;
#8610=EDGE_CURVE ( 'NONE', #23183, #62091, #71488, .T. ) ;
#8611=DIRECTION ( 'NONE',  ( 0.000000000000000000, 1.000000000000000000, 0.000000000000000000 ) ) ;
#8612=ORIENTED_EDGE ( 'NONE', *, *, #64801, .T. ) ;
#8613=EDGE_LOOP ( 'NONE', ( #2891, #61345, #125870, #11666 ) ) ;
#8614=EDGE_CURVE ( 'NONE', #96017, #127371, #69330, .T. ) ;
#8615=ADVANCED_FACE ( 'NONE', ( #112252 ), #58891, .T. ) ;
#8616=DIRECTION ( 'NONE',  ( 0.000000000000000000, 0.000000000000000000, 1.000000000000000000 ) ) ;
#8617=EDGE_CURVE ( 'NONE', #128383, #96759, #110311, .T. ) ;
#8618=VERTEX_POINT ( 'NONE', #22602 ) ;
#8619=DIRECTION ( 'NONE',  ( -4.274815082592931898E-19, -0.9999939076577903929, -0.003490651415223739937 ) ) ;
#8620=AXIS2_PLACEMENT_3D ( 'NONE', #79163, #16329, #126314 ) ;
#8622=AXIS2_PLACEMENT_3D ( 'NONE', #39557, #21161, #19216 ) ;
#8624=ORIENTED_EDGE ( 'NONE', *, *, #57574, .T. ) ;
#8626=CARTESIAN_POINT ( 'NONE',  ( -7.300000000000018474, 12.50000000000000000, -3.918623584224389056 ) ) ;
#8627=EDGE_CURVE ( 'NONE', #98294, #95448, #113259, .T. ) ;
#8629=CARTESIAN_POINT ( 'NONE',  ( -13.29999999999998828, 2.500000000000000000, 4.230127018922196669 ) ) ;
#8630=EDGE_LOOP ( 'NONE', ( #91027, #77369, #3674, #80074 ) ) ;
#8631=EDGE_CURVE ( 'NONE', #105260, #8138, #90007, .T. ) ;
#8632=CONICAL_SURFACE ( 'NONE', #50504, 0.09999999999999982514, 0.003490658503988666988 ) ;
#8633=FACE_OUTER_BOUND ( 'NONE', #47665, .T. ) ;
#8634=ORIENTED_EDGE ( 'NONE', *, *, #9047, .T. ) ;
#8635=PLANE ( 'NONE',  #17159 ) ;
#8636=CARTESIAN_POINT ( 'NONE',  ( -6.850000000000017408, 2.500000000000000000, -6.841600689897077814 ) ) ;
#8637=DIRECTION ( 'NONE',  ( 0.000000000000000000, 0.000000000000000000, 1.000000000000000000 ) ) ;
#8638=AXIS2_PLACEMENT_3D ( 'NONE', #87526, #427, #127469 ) ;
#8639=CIRCLE ( 'NONE', #81814, 0.1000000000000000472 ) ;
#8640=ORIENTED_EDGE ( 'NONE', *, *, #85471, .T. ) ;
#8641=DIRECTION ( 'NONE',  ( 0.000000000000000000, 0.000000000000000000, 1.000000000000000000 ) ) ;
#8642=VECTOR ( 'NONE', #111006, 1000.000000000000000 ) ;
#8643=EDGE_LOOP ( 'NONE', ( #55002, #87651, #59079, #66352 ) ) ;
#8644=DIRECTION ( 'NONE',  ( 0.000000000000000000, 0.000000000000000000, 1.000000000000000000 ) ) ;
#8645=DIRECTION ( 'NONE',  ( 0.000000000000000000, 0.000000000000000000, 1.000000000000000000 ) ) ;
#8646=AXIS2_PLACEMENT_3D ( 'NONE', #114278, #95934, #54699 ) ;
#8647=CARTESIAN_POINT ( 'NONE',  ( -12.09999999999999609, 12.50000000000000000, -4.330127018922198978 ) ) ;
#8648=ORIENTED_EDGE ( 'NONE', *, *, #41160, .T. ) ;
#8649=DIRECTION ( 'NONE',  ( 0.000000000000000000, -0.000000000000000000, 1.000000000000000000 ) ) ;
#8650=DIRECTION ( 'NONE',  ( -0.000000000000000000, -1.000000000000000000, -0.000000000000000000 ) ) ;
#8651=AXIS2_PLACEMENT_3D ( 'NONE', #6962, #65905, #107110 ) ;
#8652=ORIENTED_EDGE ( 'NONE', *, *, #36983, .T. ) ;
#8653=DIRECTION ( 'NONE',  ( -0.000000000000000000, -1.000000000000000000, -0.000000000000000000 ) ) ;
#8654=VERTEX_POINT ( 'NONE', #21952 ) ;
#8655=DIRECTION ( 'NONE',  ( 0.000000000000000000, 1.000000000000000000, 0.000000000000000000 ) ) ;
#8656=EDGE_CURVE ( 'NONE', #47134, #93656, #6617, .T. ) ;
#8657=ORIENTED_EDGE ( 'NONE', *, *, #48864, .T. ) ;
#8658=CARTESIAN_POINT ( 'NONE',  ( 12.89999999999990088, 2.500000000000000000, 4.430127018922196847 ) ) ;
#8659=CARTESIAN_POINT ( 'NONE',  ( -6.050000000000017586, 12.50000000000000000, 1.753560074763284016 ) ) ;
#8661=VERTEX_POINT ( 'NONE', #11462 ) ;
#8662=EDGE_LOOP ( 'NONE', ( #79028, #23814, #108464, #32036 ) ) ;
#8663=LINE ( 'NONE', #127194, #128283 ) ;
#8664=DIRECTION ( 'NONE',  ( 0.000000000000000000, 1.000000000000000000, 0.000000000000000000 ) ) ;
#8665=ORIENTED_EDGE ( 'NONE', *, *, #66679, .F. ) ;
#8666=CARTESIAN_POINT ( 'NONE',  ( -12.69999999999999396, 2.500000000000000000, 0.3464101615137776813 ) ) ;
#8667=CARTESIAN_POINT ( 'NONE',  ( -7.700000000000010836, 2.500000000000000000, 3.983716857408420964 ) ) ;
#8668=DIRECTION ( 'NONE',  ( -0.000000000000000000, 1.000000000000000000, -0.000000000000000000 ) ) ;
#8669=VECTOR ( 'NONE', #128143, 1000.000000000000000 ) ;
#8671=LINE ( 'NONE', #17192, #78165 ) ;
#8672=AXIS2_PLACEMENT_3D ( 'NONE', #46285, #87489, #17460 ) ;
#8673=VECTOR ( 'NONE', #20528, 1000.000000000000000 ) ;
#8674=CARTESIAN_POINT ( 'NONE',  ( 4.399999999999940847, 2.500000000000000000, -4.776537180435977525 ) ) ;
#8675=DIRECTION ( 'NONE',  ( 0.000000000000000000, 0.000000000000000000, -1.000000000000000000 ) ) ;
#8676=CONICAL_SURFACE ( 'NONE', #2423, 0.1000000000000002554, 0.003490658503988666988 ) ;
#8677=ORIENTED_EDGE ( 'NONE', *, *, #93318, .F. ) ;
#8678=CIRCLE ( 'NONE', #102691, 0.06509327318403745899 ) ;
#8679=EDGE_LOOP ( 'NONE', ( #96736, #79112, #68934, #100287 ) ) ;
#8680=EDGE_LOOP ( 'NONE', ( #89388, #37217 ) ) ;
#8681=ORIENTED_EDGE ( 'NONE', *, *, #128325, .T. ) ;
#8682=LINE ( 'NONE', #78102, #39177 ) ;
#8683=DIRECTION ( 'NONE',  ( 0.000000000000000000, 1.000000000000000000, 0.000000000000000000 ) ) ;
#8684=VECTOR ( 'NONE', #86795, 1000.000000000000000 ) ;
#8685=LINE ( 'NONE', #48639, #42703 ) ;
#8686=ORIENTED_EDGE ( 'NONE', *, *, #118244, .F. ) ;
#8687=FACE_BOUND ( 'NONE', #107867, .T. ) ;
#8688=ORIENTED_EDGE ( 'NONE', *, *, #108689, .T. ) ;
#8689=CARTESIAN_POINT ( 'NONE',  ( -6.850000000000013856, 12.50000000000000000, 6.213873640053559022 ) ) ;
#8690=FACE_OUTER_BOUND ( 'NONE', #17826, .T. ) ;
#8691=AXIS2_PLACEMENT_3D ( 'NONE', #57975, #48805, #97883 ) ;
#8692=DIRECTION ( 'NONE',  ( 0.000000000000000000, -0.9999939076577903929, 0.003490651415223739937 ) ) ;
#8693=DIRECTION ( 'NONE',  ( -0.000000000000000000, 1.000000000000000000, -0.000000000000000000 ) ) ;
#8694=LINE ( 'NONE', #86629, #51400 ) ;
#8695=CARTESIAN_POINT ( 'NONE',  ( -13.34999999999999076, 2.500000000000000000, 2.065063509461101621 ) ) ;
#8696=CARTESIAN_POINT ( 'NONE',  ( 2.099999999999948574, 2.500000000000000000, 4.230127018922196669 ) ) ;
#8697=CARTESIAN_POINT ( 'NONE',  ( -0.4500000000000402012, 2.500000000000000000, 6.595190528383296780 ) ) ;
#8698=DIRECTION ( 'NONE',  ( 0.000000000000000000, 0.000000000000000000, 1.000000000000000000 ) ) ;
#8699=FACE_OUTER_BOUND ( 'NONE', #67664, .T. ) ;
#8700=EDGE_CURVE ( 'NONE', #74521, #80440, #30486, .T. ) ;
#8701=EDGE_LOOP ( 'NONE', ( #59558, #62667 ) ) ;
#8702=ORIENTED_EDGE ( 'NONE', *, *, #53412, .F. ) ;
#8703=ORIENTED_EDGE ( 'NONE', *, *, #27520, .T. ) ;
#8704=EDGE_LOOP ( 'NONE', ( #70978, #52290 ) ) ;
#8705=DIRECTION ( 'NONE',  ( -0.000000000000000000, -1.000000000000000000, -0.000000000000000000 ) ) ;
#8706=B_SPLINE_CURVE_WITH_KNOTS ( 'NONE', 3,
 ( #104825, #15149, #30494, #40961, #80867, #31135, #71040, #21284, #61221, #101148, #11468, #36115 ),
 .UNSPECIFIED., .F., .F.,
 ( 4, 2, 2, 2, 2, 4 ),
 ( 0.000000000000000000, 0.001300228439403514720, 0.002600456878807029439, 0.003900685318210543942, 0.004550799537912301844, 0.005200913757614058879 ),
 .UNSPECIFIED. ) ;
#8707=CARTESIAN_POINT ( 'NONE',  ( 15.59999999999988951, 2.500000000000000000, -0.3464101615137783474 ) ) ;
#8708=ORIENTED_EDGE ( 'NONE', *, *, #75077, .F. ) ;
#8709=EDGE_LOOP ( 'NONE', ( #68552, #21572 ) ) ;
#8710=ORIENTED_EDGE ( 'NONE', *, *, #61674, .T. ) ;
#8711=DIRECTION ( 'NONE',  ( 0.000000000000000000, 1.000000000000000000, 0.000000000000000000 ) ) ;
#8712=AXIS2_PLACEMENT_3D ( 'NONE', #60795, #29409, #100703 ) ;
#8713=EDGE_CURVE ( 'NONE', #64779, #121936, #106982, .T. ) ;
#8714=PLANE ( 'NONE',  #128221 ) ;
#8715=FACE_OUTER_BOUND ( 'NONE', #121087, .T. ) ;
#8716=DIRECTION ( 'NONE',  ( 0.000000000000000000, 1.000000000000000000, 0.000000000000000000 ) ) ;
#8717=CARTESIAN_POINT ( 'NONE',  ( -5.400000000000019895, 2.500000000000000000, -0.6928203230275541413 ) ) ;
#8718=CARTESIAN_POINT ( 'NONE',  ( 0.3999999999999628852, 2.500000000000000000, 0.5928203230275517210 ) ) ;
#8719=ADVANCED_FACE ( 'NONE', ( #92608 ), #23362, .T. ) ;
#8720=DIRECTION ( 'NONE',  ( 0.000000000000000000, 1.000000000000000000, 0.000000000000000000 ) ) ;
#8721=ADVANCED_FACE ( 'NONE', ( #1002 ), #102781, .T. ) ;
#8722=EDGE_LOOP ( 'NONE', ( #24846, #16195 ) ) ;
#8723=AXIS2_PLACEMENT_3D ( 'NONE', #94957, #5894, #45209 ) ;
#8724=AXIS2_PLACEMENT_3D ( 'NONE', #90033, #120797, #41619 ) ;
#8725=DIRECTION ( 'NONE',  ( 0.000000000000000000, -0.9999939076577903929, 0.003490651415223739937 ) ) ;
#8726=ORIENTED_EDGE ( 'NONE', *, *, #118709, .F. ) ;
#8727=VERTEX_POINT ( 'NONE', #12104 ) ;
#8728=CONICAL_SURFACE ( 'NONE', #37990, 0.09999999999999999167, 0.003490658503988666988 ) ;
#8729=ORIENTED_EDGE ( 'NONE', *, *, #5321, .T. ) ;
#8730=AXIS2_PLACEMENT_3D ( 'NONE', #65553, #73431, #36105 ) ;
#8731=DIRECTION ( 'NONE',  ( 0.000000000000000000, 0.000000000000000000, 1.000000000000000000 ) ) ;
#8732=VERTEX_POINT ( 'NONE', #31763 ) ;
#8733=EDGE_CURVE ( 'NONE', #4409, #71397, #12734, .T. ) ;
#8734=EDGE_LOOP ( 'NONE', ( #123850, #4764 ) ) ;
#8736=DIRECTION ( 'NONE',  ( 0.000000000000000000, 0.000000000000000000, -1.000000000000000000 ) ) ;
#8737=AXIS2_PLACEMENT_3D ( 'NONE', #94474, #55846, #72918 ) ;
#8738=DIRECTION ( 'NONE',  ( 0.000000000000000000, 0.000000000000000000, -1.000000000000000000 ) ) ;
#8739=DIRECTION ( 'NONE',  ( 0.000000000000000000, 0.000000000000000000, 1.000000000000000000 ) ) ;
#8740=FACE_OUTER_BOUND ( 'NONE', #118935, .T. ) ;
#8741=VECTOR ( 'NONE', #75485, 1000.000000000000000 ) ;
#8742=AXIS2_PLACEMENT_3D ( 'NONE', #62382, #102301, #60461 ) ;
#8743=DIRECTION ( 'NONE',  ( 0.000000000000000000, 1.000000000000000000, 0.000000000000000000 ) ) ;
#8744=VECTOR ( 'NONE', #82759, 1000.000000000000000 ) ;
#8745=EDGE_LOOP ( 'NONE', ( #103824, #55372 ) ) ;
#8746=CARTESIAN_POINT ( 'NONE',  ( -11.64999999999999680, 2.500000000000000000, -2.165063509461097713 ) ) ;
#8747=VERTEX_POINT ( 'NONE', #91315 ) ;
#8748=DIRECTION ( 'NONE',  ( -0.000000000000000000, -1.000000000000000000, -0.000000000000000000 ) ) ;
#8749=ORIENTED_EDGE ( 'NONE', *, *, #13825, .F. ) ;
#8751=CIRCLE ( 'NONE', #60993, 0.1000000000000002554 ) ;
#8752=DIRECTION ( 'NONE',  ( -0.000000000000000000, -1.000000000000000000, -0.000000000000000000 ) ) ;
#8753=B_SPLINE_CURVE_WITH_KNOTS ( 'NONE', 3,
 ( #126159, #96050, #65289, #46298, #16815, #115684, #74485, #85586 ),
 .UNSPECIFIED., .F., .F.,
 ( 4, 2, 2, 4 ),
 ( 0.002994103107820000886, 0.003957537843903918655, 0.004920972579987836423, 0.006847842052155671960 ),
 .UNSPECIFIED. ) ;
#8754=ORIENTED_EDGE ( 'NONE', *, *, #57411, .F. ) ;
#8755=CARTESIAN_POINT ( 'NONE',  ( 8.749999999999920064, 2.500000000000000000, -2.757883832488654097 ) ) ;
#8756=CARTESIAN_POINT ( 'NONE',  ( 9.599999999999914380, 2.500000000000000000, 5.122947341949749323 ) ) ;
#8757=VERTEX_POINT ( 'NONE', #10789 ) ;
#8758=ADVANCED_FACE ( 'NONE', ( #52679 ), #46353, .T. ) ;
#8759=CARTESIAN_POINT ( 'NONE',  ( -15.39999999999998082, 2.500000000000000000, 0.5928203230275517210 ) ) ;
#8760=ORIENTED_EDGE ( 'NONE', *, *, #51701, .F. ) ;
#8761=EDGE_LOOP ( 'NONE', ( #40648, #78146, #111751, #45036 ) ) ;
#8762=DIRECTION ( 'NONE',  ( 0.000000000000000000, 0.000000000000000000, 1.000000000000000000 ) ) ;
#8763=DIRECTION ( 'NONE',  ( 0.000000000000000000, 0.000000000000000000, 1.000000000000000000 ) ) ;
#8764=EDGE_CURVE ( 'NONE', #55169, #87449, #96512, .T. ) ;
#8766=CARTESIAN_POINT ( 'NONE',  ( 9.149999999999920419, 12.50000000000000000, 1.472243186433545459 ) ) ;
#8767=ADVANCED_FACE ( 'NONE', ( #90665 ), #88102, .T. ) ;
#8768=CARTESIAN_POINT ( 'NONE',  ( 1.849999999999949685, 12.50000000000000000, 1.818653347947321475 ) ) ;
#8769=ORIENTED_EDGE ( 'NONE', *, *, #103114, .F. ) ;
#8770=LINE ( 'NONE', #10086, #36290 ) ;
#8771=CIRCLE ( 'NONE', #15019, 0.1000000000000002554 ) ;
#8772=CIRCLE ( 'NONE', #27638, 0.1000000000000002554 ) ;
#8773=ADVANCED_FACE ( 'NONE', ( #110937 ), #25510, .T. ) ;
#8774=VECTOR ( 'NONE', #70115, 1000.000000000000000 ) ;
#8775=EDGE_CURVE ( 'NONE', #43807, #53996, #104842, .T. ) ;
#8776=ADVANCED_FACE ( 'NONE', ( #14027 ), #74259, .T. ) ;
#8777=EDGE_CURVE ( 'NONE', #109700, #81402, #27651, .T. ) ;
#8778=VERTEX_POINT ( 'NONE', #63144 ) ;
#8779=CARTESIAN_POINT ( 'NONE',  ( 0.6499999999999561684, 2.500000000000000000, 2.511473670974873507 ) ) ;
#8780=DIRECTION ( 'NONE',  ( -0.000000000000000000, 1.000000000000000000, -0.000000000000000000 ) ) ;
#8781=AXIS2_PLACEMENT_3D ( 'NONE', #127480, #75157, #26697 ) ;
#8782=AXIS2_PLACEMENT_3D ( 'NONE', #72075, #83178, #32153 ) ;
#8783=VECTOR ( 'NONE', #82813, 1000.000000000000000 ) ;
#8784=ORIENTED_EDGE ( 'NONE', *, *, #13776, .T. ) ;
#8785=ADVANCED_FACE ( 'NONE', ( #63801 ), #96610, .T. ) ;
#8786=AXIS2_PLACEMENT_3D ( 'NONE', #25144, #115440, #6143 ) ;
#8787=CIRCLE ( 'NONE', #121666, 0.06509327318403745899 ) ;
#8788=CARTESIAN_POINT ( 'NONE',  ( 7.699999999999923794, 2.500000000000000000, -0.4464101615137783252 ) ) ;
#8789=CARTESIAN_POINT ( 'NONE',  ( 8.549999999999922551, 2.500000000000000000, 2.511473670974873507 ) ) ;
#8790=DIRECTION ( 'NONE',  ( 0.000000000000000000, 0.000000000000000000, 1.000000000000000000 ) ) ;
#8791=CARTESIAN_POINT ( 'NONE',  ( -11.64999999999999680, 12.50000000000000000, -2.922977105672687426 ) ) ;
#8792=PLANE ( 'NONE',  #70436 ) ;
#8793=ORIENTED_EDGE ( 'NONE', *, *, #58941, .T. ) ;
#8794=EDGE_CURVE ( 'NONE', #103548, #76584, #92419, .T. ) ;
#8795=VECTOR ( 'NONE', #83647, 1000.000000000000000 ) ;
#8796=FACE_OUTER_BOUND ( 'NONE', #3440, .T. ) ;
#8797=DIRECTION ( 'NONE',  ( 0.000000000000000000, 0.000000000000000000, 1.000000000000000000 ) ) ;
#8798=ORIENTED_EDGE ( 'NONE', *, *, #120900, .F. ) ;
#8799=CARTESIAN_POINT ( 'NONE',  ( -8.950000000000008171, 2.500000000000000000, -2.511473670974877948 ) ) ;
#8800=ORIENTED_EDGE ( 'NONE', *, *, #6353, .T. ) ;
#8801=ORIENTED_EDGE ( 'NONE', *, *, #63503, .F. ) ;
#8803=ORIENTED_EDGE ( 'NONE', *, *, #63561, .T. ) ;
#8805=CARTESIAN_POINT ( 'NONE',  ( -6.050000000000017586, 2.500000000000000000, 1.718653347947321386 ) ) ;
#8806=CIRCLE ( 'NONE', #17104, 0.06509327318403745899 ) ;
#8807=EDGE_LOOP ( 'NONE', ( #72916, #792, #68472, #109596 ) ) ;
#8808=DIRECTION ( 'NONE',  ( 0.000000000000000000, 0.000000000000000000, -1.000000000000000000 ) ) ;
#8809=DIRECTION ( 'NONE',  ( -0.000000000000000000, -1.000000000000000000, -0.000000000000000000 ) ) ;
#8810=ORIENTED_EDGE ( 'NONE', *, *, #95497, .T. ) ;
#8812=FACE_OUTER_BOUND ( 'NONE', #43255, .T. ) ;
#8813=AXIS2_PLACEMENT_3D ( 'NONE', #31222, #91410, #122175 ) ;
#8814=ORIENTED_EDGE ( 'NONE', *, *, #20669, .T. ) ;
#8815=CIRCLE ( 'NONE', #48557, 0.1000000000000002554 ) ;
#8816=AXIS2_PLACEMENT_3D ( 'NONE', #125800, #106810, #17114 ) ;
#8817=AXIS2_PLACEMENT_3D ( 'NONE', #73030, #23942, #66267 ) ;
#8818=EDGE_CURVE ( 'NONE', #4150, #7088, #4852, .T. ) ;
#8819=VERTEX_POINT ( 'NONE', #113532 ) ;
#8820=EDGE_LOOP ( 'NONE', ( #117894, #46706 ) ) ;
#8821=CARTESIAN_POINT ( 'NONE',  ( -4.600000000000024514, 2.500000000000000000, -0.6928203230275542523 ) ) ;
#8822=DIRECTION ( 'NONE',  ( 0.000000000000000000, -0.9999939076577903929, 0.003490651415223739937 ) ) ;
#8823=DIRECTION ( 'NONE',  ( 0.000000000000000000, -0.000000000000000000, 1.000000000000000000 ) ) ;
#8824=FACE_BOUND ( 'NONE', #57735, .T. ) ;
#8825=ORIENTED_EDGE ( 'NONE', *, *, #5774, .F. ) ;
#8826=CARTESIAN_POINT ( 'NONE',  ( 5.849999999999932143, 2.500000000000000000, 2.065063509461097624 ) ) ;
#8827=CARTESIAN_POINT ( 'NONE',  ( -0.6000000000000383915, 2.500000000000000000, -4.676537180435977881 ) ) ;
#8829=ORIENTED_EDGE ( 'NONE', *, *, #59469, .T. ) ;
#8830=CIRCLE ( 'NONE', #6758, 0.1000000000000002554 ) ;
#8831=ADVANCED_FACE ( 'NONE', ( #85360 ), #56894, .T. ) ;
#8832=LINE ( 'NONE', #48785, #117620 ) ;
#8833=PLANE ( 'NONE',  #11542 ) ;
#8834=AXIS2_PLACEMENT_3D ( 'NONE', #91028, #111967, #58 ) ;
#8835=VECTOR ( 'NONE', #24354, 1000.000000000000000 ) ;
#8836=FACE_OUTER_BOUND ( 'NONE', #78661, .T. ) ;
#8837=CARTESIAN_POINT ( 'NONE',  ( 8.349999999999919709, 12.50000000000000000, -1.537336459617587581 ) ) ;
#8838=FACE_OUTER_BOUND ( 'NONE', #87394, .T. ) ;
#8839=DIRECTION ( 'NONE',  ( 0.000000000000000000, 1.000000000000000000, 0.000000000000000000 ) ) ;
#8840=AXIS2_PLACEMENT_3D ( 'NONE', #88355, #128323, #51690 ) ;
#8841=DIRECTION ( 'NONE',  ( -0.000000000000000000, 1.000000000000000000, -0.000000000000000000 ) ) ;
#8842=VERTEX_POINT ( 'NONE', #125916 ) ;
#8843=CIRCLE ( 'NONE', #46503, 0.1000000000000002554 ) ;
#8844=VERTEX_POINT ( 'NONE', #55894 ) ;
#8845=EDGE_LOOP ( 'NONE', ( #96616, #61863, #98127, #52050 ) ) ;
#8846=ORIENTED_EDGE ( 'NONE', *, *, #116653, .T. ) ;
#8847=ORIENTED_EDGE ( 'NONE', *, *, #69404, .F. ) ;
#8848=CARTESIAN_POINT ( 'NONE',  ( -8.150000000000012790, 12.50000000000000000, -1.818653347947326138 ) ) ;
#8849=DIRECTION ( 'NONE',  ( -0.000000000000000000, 1.000000000000000000, -0.000000000000000000 ) ) ;
#8850=ORIENTED_EDGE ( 'NONE', *, *, #2427, .T. ) ;
#8851=FACE_BOUND ( 'NONE', #69460, .T. ) ;
#8852=FACE_OUTER_BOUND ( 'NONE', #46664, .T. ) ;
#8853=CARTESIAN_POINT ( 'NONE',  ( -8.550000000000011369, 12.50000000000000000, 1.883746621131358934 ) ) ;
#8854=DIRECTION ( 'NONE',  ( 0.000000000000000000, 0.000000000000000000, 1.000000000000000000 ) ) ;
#8855=FACE_OUTER_BOUND ( 'NONE', #62365, .T. ) ;
#8856=DIRECTION ( 'NONE',  ( 0.000000000000000000, 0.000000000000000000, 1.000000000000000000 ) ) ;
#8857=ORIENTED_EDGE ( 'NONE', *, *, #87078, .T. ) ;
#8858=EDGE_LOOP ( 'NONE', ( #113677, #10481 ) ) ;
#8859=EDGE_LOOP ( 'NONE', ( #64817, #71563 ) ) ;
#8860=AXIS2_PLACEMENT_3D ( 'NONE', #15428, #29157, #101099 ) ;
#8861=EDGE_LOOP ( 'NONE', ( #33621, #107525, #11255, #65914 ) ) ;
#8862=CIRCLE ( 'NONE', #2606, 0.06509327318403745899 ) ;
#8863=CARTESIAN_POINT ( 'NONE',  ( -1.650000000000034772, 12.50000000000000000, 6.560283801567334372 ) ) ;
#8864=CIRCLE ( 'NONE', #557, 0.06509327318403745899 ) ;
#8865=CARTESIAN_POINT ( 'NONE',  ( 4.999999999999938716, 12.50000000000000000, -5.022947341949754119 ) ) ;
#8866=CARTESIAN_POINT ( 'NONE',  ( -5.400000000000024336, 2.500000000000000000, -3.637306695894650055 ) ) ;
#8867=ORIENTED_EDGE ( 'NONE', *, *, #121327, .F. ) ;
#8868=DIRECTION ( 'NONE',  ( 0.000000000000000000, 0.000000000000000000, -1.000000000000000000 ) ) ;
#8869=EDGE_CURVE ( 'NONE', #122246, #46899, #4655, .T. ) ;
#8870=LINE ( 'NONE', #39032, #36546 ) ;
#8871=CONICAL_SURFACE ( 'NONE', #25591, 0.09999999999999982514, 0.003490658503988666988 ) ;
#8872=AXIS2_PLACEMENT_3D ( 'NONE', #95415, #105228, #97340 ) ;
#8873=CIRCLE ( 'NONE', #25594, 0.1000000000000002554 ) ;
#8874=DIRECTION ( 'NONE',  ( 0.000000000000000000, -0.9999939076577903929, 0.003490651415223739937 ) ) ;
#8876=DIRECTION ( 'NONE',  ( -0.000000000000000000, -1.000000000000000000, -0.000000000000000000 ) ) ;
#8877=CARTESIAN_POINT ( 'NONE',  ( 11.24999999999994493, 2.500000000000000000, 6.495190528383297135 ) ) ;
#8878=AXIS2_PLACEMENT_3D ( 'NONE', #91165, #22447, #59803 ) ;
#8879=ADVANCED_FACE ( 'NONE', ( #94531 ), #93903, .T. ) ;
#8880=CIRCLE ( 'NONE', #59077, 0.1000000000000002554 ) ;
#8881=EDGE_CURVE ( 'NONE', #88669, #128715, #7356, .T. ) ;
#8882=DIRECTION ( 'NONE',  ( 0.000000000000000000, -0.000000000000000000, 1.000000000000000000 ) ) ;
#8883=ADVANCED_FACE ( 'NONE', ( #124650 ), #86141, .T. ) ;
#8884=ORIENTED_EDGE ( 'NONE', *, *, #83856, .T. ) ;
#8885=CARTESIAN_POINT ( 'NONE',  ( 14.14999999999989377, 12.50000000000000000, -2.922977105672691422 ) ) ;
#8886=AXIS2_PLACEMENT_3D ( 'NONE', #48225, #50178, #57407 ) ;
#8887=ORIENTED_EDGE ( 'NONE', *, *, #13023, .F. ) ;
#8888=ORIENTED_EDGE ( 'NONE', *, *, #115363, .F. ) ;
#8889=DIRECTION ( 'NONE',  ( 0.000000000000000000, 1.000000000000000000, 0.000000000000000000 ) ) ;
#8890=EDGE_CURVE ( 'NONE', #7809, #65690, #107081, .T. ) ;
#8891=DIRECTION ( 'NONE',  ( -0.000000000000000000, 1.000000000000000000, -0.000000000000000000 ) ) ;
#8892=DIRECTION ( 'NONE',  ( 0.000000000000000000, -0.000000000000000000, 1.000000000000000000 ) ) ;
#8893=EDGE_CURVE ( 'NONE', #67022, #69080, #73635, .T. ) ;
#8894=ORIENTED_EDGE ( 'NONE', *, *, #114161, .T. ) ;
#8895=EDGE_LOOP ( 'NONE', ( #31628, #102122, #108395, #118547 ) ) ;
#8896=AXIS2_PLACEMENT_3D ( 'NONE', #126007, #116189, #26533 ) ;
#8897=CARTESIAN_POINT ( 'NONE',  ( 5.399999999999936406, 2.500000000000000000, -3.537306695894649966 ) ) ;
#8898=FACE_OUTER_BOUND ( 'NONE', #28262, .T. ) ;
#8899=EDGE_LOOP ( 'NONE', ( #77896, #127489 ) ) ;
#8900=EDGE_LOOP ( 'NONE', ( #55225, #38942 ) ) ;
#8901=CARTESIAN_POINT ( 'NONE',  ( 0.8499999999999557909, 2.500000000000000000, -7.288010851410854585 ) ) ;
#8902=CIRCLE ( 'NONE', #79928, 0.06509327318403745899 ) ;
#8903=EDGE_LOOP ( 'NONE', ( #44443, #62662 ) ) ;
#8904=DIRECTION ( 'NONE',  ( 0.000000000000000000, 0.000000000000000000, 1.000000000000000000 ) ) ;
#8905=AXIS2_PLACEMENT_3D ( 'NONE', #46857, #86760, #75021 ) ;
#8906=AXIS2_PLACEMENT_3D ( 'NONE', #122533, #70850, #93710 ) ;
#8907=ORIENTED_EDGE ( 'NONE', *, *, #61142, .T. ) ;
#8908=DIRECTION ( 'NONE',  ( 0.000000000000000000, 0.000000000000000000, 1.000000000000000000 ) ) ;
#8909=DIRECTION ( 'NONE',  ( -0.000000000000000000, -1.000000000000000000, -0.000000000000000000 ) ) ;
#8910=CARTESIAN_POINT ( 'NONE',  ( 1.649999999999950617, 2.500000000000000000, 2.165063509461097713 ) ) ;
#8911=CARTESIAN_POINT ( 'NONE',  ( 1.649999999999950617, 12.50000000000000000, 2.230156782645134950 ) ) ;
#8912=ORIENTED_EDGE ( 'NONE', *, *, #55033, .F. ) ;
#8913=CONICAL_SURFACE ( 'NONE', #98801, 0.1000000000000000472, 0.003490658503988666988 ) ;
#8914=AXIS2_PLACEMENT_3D ( 'NONE', #120611, #61706, #30318 ) ;
#8915=DIRECTION ( 'NONE',  ( 0.000000000000000000, 0.000000000000000000, 1.000000000000000000 ) ) ;
#8916=AXIS2_PLACEMENT_3D ( 'NONE', #4114, #74811, #42805 ) ;
#8917=ORIENTED_EDGE ( 'NONE', *, *, #71459, .F. ) ;
#8918=ORIENTED_EDGE ( 'NONE', *, *, #36264, .F. ) ;
#8919=DIRECTION ( 'NONE',  ( 0.000000000000000000, 1.000000000000000000, 0.000000000000000000 ) ) ;
#8920=LINE ( 'NONE', #96652, #67926 ) ;
#8921=LINE ( 'NONE', #39074, #40702 ) ;
#8922=CARTESIAN_POINT ( 'NONE',  ( -1.450000000000035483, 2.500000000000000000, 6.248780366869521430 ) ) ;
#8923=CIRCLE ( 'NONE', #125994, 0.06509327318403745899 ) ;
#8924=CARTESIAN_POINT ( 'NONE',  ( 8.099999999999921485, 12.50000000000000000, 0.4115034346978109769 ) ) ;
#8925=DIRECTION ( 'NONE',  ( 0.000000000000000000, 0.000000000000000000, -1.000000000000000000 ) ) ;
#8926=DIRECTION ( 'NONE',  ( -0.000000000000000000, -1.000000000000000000, -0.000000000000000000 ) ) ;
#8927=CARTESIAN_POINT ( 'NONE',  ( -8.749999999999976907, 2.500000000000000000, -6.595190528383296780 ) ) ;
#8928=AXIS2_PLACEMENT_3D ( 'NONE', #73282, #102111, #70712 ) ;
#8929=CARTESIAN_POINT ( 'NONE',  ( 3.149999999999942624, 12.50000000000000000, 6.148780366869520897 ) ) ;
#8930=ADVANCED_FACE ( 'NONE', ( #65716 ), #105655, .T. ) ;
#8931=ADVANCED_FACE ( 'NONE', ( #54594 ), #44807, .T. ) ;
#8932=AXIS2_PLACEMENT_3D ( 'NONE', #23496, #73893, #94175 ) ;
#8933=EDGE_CURVE ( 'NONE', #81692, #44808, #17174, .T. ) ;
#8934=CARTESIAN_POINT ( 'NONE',  ( 8.299999999999922551, 2.500000000000000000, 0.09999999999999761857 ) ) ;
#8936=ORIENTED_EDGE ( 'NONE', *, *, #74247, .T. ) ;
#8937=EDGE_CURVE ( 'NONE', #78082, #33468, #63186, .T. ) ;
#8938=DIRECTION ( 'NONE',  ( 0.000000000000000000, 0.000000000000000000, 1.000000000000000000 ) ) ;
#8939=DIRECTION ( 'NONE',  ( -4.274815082592931898E-19, -0.9999939076577903929, -0.003490651415223739937 ) ) ;
#8940=DIRECTION ( 'NONE',  ( 0.000000000000000000, 0.000000000000000000, 1.000000000000000000 ) ) ;
#8941=CARTESIAN_POINT ( 'NONE',  ( -9.400000000000007461, 12.50000000000000000, 4.048810130592458201 ) ) ;
#8942=FACE_OUTER_BOUND ( 'NONE', #8280, .T. ) ;
#8943=ORIENTED_EDGE ( 'NONE', *, *, #49298, .F. ) ;
#8944=EDGE_CURVE ( 'NONE', #52806, #113778, #67349, .T. ) ;
#8945=CARTESIAN_POINT ( 'NONE',  ( -14.99999999999998401, 12.50000000000000000, 0.6277270498435143509 ) ) ;
#8946=EDGE_CURVE ( 'NONE', #112348, #7603, #48609, .T. ) ;
#8947=CARTESIAN_POINT ( 'NONE',  ( 1.249999999999954259, 12.50000000000000000, -7.188010851410854052 ) ) ;
#8948=CARTESIAN_POINT ( 'NONE',  ( 4.599999999999940137, 2.500000000000000000, -5.022947341949754119 ) ) ;
#8949=VERTEX_POINT ( 'NONE', #58503 ) ;
#8950=VECTOR ( 'NONE', #16961, 1000.000000000000000 ) ;
#8951=EDGE_CURVE ( 'NONE', #94541, #96192, #78131, .T. ) ;
#8953=CARTESIAN_POINT ( 'NONE',  ( -9.800000000000006040, 12.50000000000000000, -4.741630453620011565 ) ) ;
#8956=ORIENTED_EDGE ( 'NONE', *, *, #19548, .T. ) ;
#8957=VECTOR ( 'NONE', #106723, 1000.000000000000000 ) ;
#8958=ORIENTED_EDGE ( 'NONE', *, *, #81101, .T. ) ;
#8959=DIRECTION ( 'NONE',  ( 0.000000000000000000, 1.000000000000000000, 0.000000000000000000 ) ) ;
#8960=CIRCLE ( 'NONE', #111468, 0.09999999999999999167 ) ;
#8961=CIRCLE ( 'NONE', #31982, 0.09999999999999982514 ) ;
#8962=CARTESIAN_POINT ( 'NONE',  ( 4.349999999999938360, 12.50000000000000000, 1.818653347947321475 ) ) ;
#8963=PLANE ( 'NONE',  #27431 ) ;
#8964=CARTESIAN_POINT ( 'NONE',  ( 7.499999999999960032, 2.500000000000000000, -0.1000000000000022815 ) ) ;
#8965=CIRCLE ( 'NONE', #128115, 0.1000000000000000472 ) ;
#8966=EDGE_LOOP ( 'NONE', ( #120547, #38560, #49456, #51909 ) ) ;
#8967=AXIS2_PLACEMENT_3D ( 'NONE', #36348, #76257, #26510 ) ;
#8968=CARTESIAN_POINT ( 'NONE',  ( 8.299999999999922551, 12.50000000000000000, -2.385244779468109755E-15 ) ) ;
#8969=AXIS2_PLACEMENT_3D ( 'NONE', #116912, #44979, #6300 ) ;
#8970=EDGE_LOOP ( 'NONE', ( #122796, #76600 ) ) ;
#8971=FACE_OUTER_BOUND ( 'NONE', #112421, .T. ) ;
#8972=CARTESIAN_POINT ( 'NONE',  ( 20.64614705759127133, -2.669560853935763589, -2.247897417623094363 ) ) ;
#8973=CIRCLE ( 'NONE', #6809, 0.1000000000000002554 ) ;
#8974=CARTESIAN_POINT ( 'NONE',  ( 17.29982614914977646, 2.489966891809544780, 2.989943721785365938 ) ) ;
#8975=DIRECTION ( 'NONE',  ( 0.000000000000000000, 0.000000000000000000, -1.000000000000000000 ) ) ;
#8976=LINE ( 'NONE', #58102, #93547 ) ;
#8977=CIRCLE ( 'NONE', #86342, 0.09999999999999982514 ) ;
#8978=VERTEX_POINT ( 'NONE', #98386 ) ;
#8979=ORIENTED_EDGE ( 'NONE', *, *, #19266, .F. ) ;
#8980=ORIENTED_EDGE ( 'NONE', *, *, #111325, .F. ) ;
#8981=ORIENTED_EDGE ( 'NONE', *, *, #33585, .T. ) ;
#8982=ORIENTED_EDGE ( 'NONE', *, *, #42656, .F. ) ;
#8983=DIRECTION ( 'NONE',  ( 0.000000000000000000, 0.000000000000000000, -1.000000000000000000 ) ) ;
#8984=CARTESIAN_POINT ( 'NONE',  ( -11.84999999999999787, 12.50000000000000000, -6.213873640053560798 ) ) ;
#8985=PLANE ( 'NONE',  #12676 ) ;
#8986=FACE_BOUND ( 'NONE', #40798, .T. ) ;
#8987=DIRECTION ( 'NONE',  ( 0.000000000000000000, 0.000000000000000000, -1.000000000000000000 ) ) ;
#8988=DIRECTION ( 'NONE',  ( 0.000000000000000000, 0.000000000000000000, 1.000000000000000000 ) ) ;
#8989=DIRECTION ( 'NONE',  ( 0.000000000000000000, 0.000000000000000000, 1.000000000000000000 ) ) ;
#8990=CARTESIAN_POINT ( 'NONE',  ( 11.64999999999990621, 12.50000000000000000, 6.430097255199259010 ) ) ;
#8991=CIRCLE ( 'NONE', #29944, 0.06509327318403745899 ) ;
#8992=EDGE_CURVE ( 'NONE', #61342, #125293, #98672, .T. ) ;
#8993=DIRECTION ( 'NONE',  ( 0.000000000000000000, 0.000000000000000000, -1.000000000000000000 ) ) ;
#8994=DIRECTION ( 'NONE',  ( 0.000000000000000000, -0.000000000000000000, 1.000000000000000000 ) ) ;
#8995=CARTESIAN_POINT ( 'NONE',  ( 12.89999999999989910, 12.50000000000000000, -0.6928203230275542523 ) ) ;
#8996=AXIS2_PLACEMENT_3D ( 'NONE', #60187, #102660, #20247 ) ;
#8997=CIRCLE ( 'NONE', #88418, 0.06509327318403741736 ) ;
#8998=CIRCLE ( 'NONE', #126075, 0.1000000000000000472 ) ;
#8999=DIRECTION ( 'NONE',  ( -0.000000000000000000, -1.000000000000000000, -0.000000000000000000 ) ) ;
#9000=VERTEX_POINT ( 'NONE', #86646 ) ;
#9001=VERTEX_POINT ( 'NONE', #116741 ) ;
#9002=ORIENTED_EDGE ( 'NONE', *, *, #126380, .T. ) ;
#9003=ORIENTED_EDGE ( 'NONE', *, *, #76254, .T. ) ;
#9004=CARTESIAN_POINT ( 'NONE',  ( -13.74999999999998757, 2.500000000000000000, 1.472243186433549456 ) ) ;
#9005=LINE ( 'NONE', #48960, #115637 ) ;
#9006=FACE_BOUND ( 'NONE', #96670, .T. ) ;
#9007=CIRCLE ( 'NONE', #119731, 0.1000000000000002554 ) ;
#9008=AXIS2_PLACEMENT_3D ( 'NONE', #113080, #41796, #122918 ) ;
#9009=DIRECTION ( 'NONE',  ( -0.000000000000000000, 1.000000000000000000, -0.000000000000000000 ) ) ;
#9010=CIRCLE ( 'NONE', #55089, 0.06509327318403745899 ) ;
#9011=CIRCLE ( 'NONE', #40344, 0.06509327318403745899 ) ;
#9012=ORIENTED_EDGE ( 'NONE', *, *, #56336, .F. ) ;
#9013=CARTESIAN_POINT ( 'NONE',  ( 1.249999999999988454, 12.50000000000000000, 2.165063509461097713 ) ) ;
#9014=DIRECTION ( 'NONE',  ( 0.000000000000000000, 0.000000000000000000, -1.000000000000000000 ) ) ;
#9015=DIRECTION ( 'NONE',  ( -0.000000000000000000, -1.000000000000000000, -0.000000000000000000 ) ) ;
#9016=EDGE_CURVE ( 'NONE', #93873, #113633, #42265, .T. ) ;
#9017=CARTESIAN_POINT ( 'NONE',  ( -6.650000000000014566, 12.50000000000000000, 2.165063509461097713 ) ) ;
#9018=ORIENTED_EDGE ( 'NONE', *, *, #67845, .F. ) ;
#9019=AXIS2_PLACEMENT_3D ( 'NONE', #7048, #65329, #66623 ) ;
#9020=PLANE ( 'NONE',  #118145 ) ;
#9021=CIRCLE ( 'NONE', #124051, 0.1000000000000000472 ) ;
#9022=CONICAL_SURFACE ( 'NONE', #59234, 0.09999999999999982514, 0.003490658503988666988 ) ;
#9023=EDGE_LOOP ( 'NONE', ( #76449, #20500, #89779, #31353 ) ) ;
#9024=ORIENTED_EDGE ( 'NONE', *, *, #104554, .F. ) ;
#9025=DIRECTION ( 'NONE',  ( 0.000000000000000000, -0.000000000000000000, 1.000000000000000000 ) ) ;
#9026=DIRECTION ( 'NONE',  ( -0.000000000000000000, 1.000000000000000000, -0.000000000000000000 ) ) ;
#9027=VERTEX_POINT ( 'NONE', #77471 ) ;
#9028=ADVANCED_FACE ( 'NONE', ( #28386 ), #75687, .T. ) ;
#9029=PLANE ( 'NONE',  #111657 ) ;
#9030=CIRCLE ( 'NONE', #92372, 0.1000000000000002554 ) ;
#9031=DIRECTION ( 'NONE',  ( -0.000000000000000000, 1.000000000000000000, -0.000000000000000000 ) ) ;
#9032=ORIENTED_EDGE ( 'NONE', *, *, #172, .T. ) ;
#9033=DIRECTION ( 'NONE',  ( 0.000000000000000000, -0.000000000000000000, 1.000000000000000000 ) ) ;
#9034=ORIENTED_EDGE ( 'NONE', *, *, #70418, .T. ) ;
#9035=ADVANCED_FACE ( 'NONE', ( #16604 ), #57847, .T. ) ;
#9036=DIRECTION ( 'NONE',  ( 0.000000000000000000, 1.000000000000000000, 0.000000000000000000 ) ) ;
#9037=EDGE_CURVE ( 'NONE', #6696, #95907, #2519, .T. ) ;
#9038=EDGE_LOOP ( 'NONE', ( #25672, #10330 ) ) ;
#9039=FACE_OUTER_BOUND ( 'NONE', #112352, .T. ) ;
#9040=FACE_BOUND ( 'NONE', #24731, .T. ) ;
#9041=ORIENTED_EDGE ( 'NONE', *, *, #121066, .F. ) ;
#9043=EDGE_LOOP ( 'NONE', ( #55633, #66768, #43056, #8867 ) ) ;
#9045=CARTESIAN_POINT ( 'NONE',  ( -5.650000000000019895, 12.50000000000000000, 1.883746621131358934 ) ) ;
#9046=ADVANCED_FACE ( 'NONE', ( #127859 ), #97755, .T. ) ;
#9047=EDGE_CURVE ( 'NONE', #46827, #70903, #69434, .T. ) ;
#9048=AXIS2_PLACEMENT_3D ( 'NONE', #105997, #77181, #45798 ) ;
#9049=CARTESIAN_POINT ( 'NONE',  ( -7.500000000000001776, -1.500000000000000000, 1.734723475976807094E-15 ) ) ;
#9050=CIRCLE ( 'NONE', #98948, 0.09999999999999982514 ) ;
#9051=EDGE_CURVE ( 'NONE', #94980, #103724, #23468, .T. ) ;
#9053=EDGE_CURVE ( 'NONE', #113165, #98051, #33940, .T. ) ;
#9054=ADVANCED_FACE ( 'NONE', ( #59137 ), #26452, .T. ) ;
#9055=FACE_OUTER_BOUND ( 'NONE', #51411, .T. ) ;
#9056=EDGE_LOOP ( 'NONE', ( #27589, #112836 ) ) ;
#9057=ORIENTED_EDGE ( 'NONE', *, *, #28914, .F. ) ;
#9058=ORIENTED_EDGE ( 'NONE', *, *, #88592, .F. ) ;
#9059=CARTESIAN_POINT ( 'NONE',  ( -9.150000000000009237, 2.500000000000000000, 1.472243186433545459 ) ) ;
#9060=AXIS2_PLACEMENT_3D ( 'NONE', #123429, #44223, #73682 ) ;
#9061=CIRCLE ( 'NONE', #126140, 0.06509327318403745899 ) ;
#9062=FACE_OUTER_BOUND ( 'NONE', #114783, .T. ) ;
#9063=CIRCLE ( 'NONE', #13260, 0.06509327318403745899 ) ;
#9064=CIRCLE ( 'NONE', #73908, 0.06509327318403745899 ) ;
#9065=DIRECTION ( 'NONE',  ( -4.274815082592931898E-19, -0.9999939076577903929, -0.003490651415223739937 ) ) ;
#9066=ORIENTED_EDGE ( 'NONE', *, *, #15107, .F. ) ;
#9067=ORIENTED_EDGE ( 'NONE', *, *, #36889, .T. ) ;
#9068=VERTEX_POINT ( 'NONE', #129186 ) ;
#9069=EDGE_CURVE ( 'NONE', #31487, #37042, #39514, .T. ) ;
#9070=LINE ( 'NONE', #20184, #127146 ) ;
#9071=CARTESIAN_POINT ( 'NONE',  ( -8.350000000000010303, 2.500000000000000000, 6.495190528383297135 ) ) ;
#9072=CIRCLE ( 'NONE', #63456, 0.06509327318403741736 ) ;
#9073=CIRCLE ( 'NONE', #4942, 0.1000000000000002554 ) ;
#9074=AXIS2_PLACEMENT_3D ( 'NONE', #59201, #118095, #68352 ) ;
#9075=CARTESIAN_POINT ( 'NONE',  ( -4.150000000000024336, 12.50000000000000000, -2.165063509461101710 ) ) ;
#9076=CARTESIAN_POINT ( 'NONE',  ( 2.099999999999950351, 2.500000000000000000, -2.276824562219559311E-15 ) ) ;
#9077=DIRECTION ( 'NONE',  ( 0.000000000000000000, 0.000000000000000000, 1.000000000000000000 ) ) ;
#9078=DIRECTION ( 'NONE',  ( 0.000000000000000000, 0.000000000000000000, 1.000000000000000000 ) ) ;
#9079=DIRECTION ( 'NONE',  ( -0.000000000000000000, -1.000000000000000000, -0.000000000000000000 ) ) ;
#9080=AXIS2_PLACEMENT_3D ( 'NONE', #68817, #7304, #28253 ) ;
#9081=LINE ( 'NONE', #56871, #22798 ) ;
#9082=CIRCLE ( 'NONE', #82254, 0.1000000000000002554 ) ;
#9083=ORIENTED_EDGE ( 'NONE', *, *, #127753, .T. ) ;
#9084=ORIENTED_EDGE ( 'NONE', *, *, #80921, .T. ) ;
#9085=DIRECTION ( 'NONE',  ( -0.000000000000000000, -1.000000000000000000, -0.000000000000000000 ) ) ;
#9086=CARTESIAN_POINT ( 'NONE',  ( -9.400000000000009237, 12.50000000000000000, -4.676537180435974328 ) ) ;
#9088=ORIENTED_EDGE ( 'NONE', *, *, #112002, .F. ) ;
#9090=DIRECTION ( 'NONE',  ( 0.000000000000000000, 1.000000000000000000, 0.000000000000000000 ) ) ;
#9091=CARTESIAN_POINT ( 'NONE',  ( 15.83209681635537258, -2.500000000000000000, 5.404881881984332281 ) ) ;
#9092=AXIS2_PLACEMENT_3D ( 'NONE', #9314, #49259, #89164 ) ;
#9093=CARTESIAN_POINT ( 'NONE',  ( -3.300000000000028244, 2.500000000000000000, 4.230127018922196669 ) ) ;
#9094=CARTESIAN_POINT ( 'NONE',  ( -13.94999999999998685, 2.500000000000000000, -2.511473670974875727 ) ) ;
#9095=DIRECTION ( 'NONE',  ( 0.000000000000000000, 1.000000000000000000, 0.000000000000000000 ) ) ;
#9096=DIRECTION ( 'NONE',  ( 0.000000000000000000, 1.000000000000000000, 0.000000000000000000 ) ) ;
#9097=EDGE_CURVE ( 'NONE', #127312, #24007, #119607, .T. ) ;
#9098=CONICAL_SURFACE ( 'NONE', #88508, 0.1000000000000002554, 0.003490658503988666988 ) ;
#9099=EDGE_CURVE ( 'NONE', #110247, #61095, #84100, .T. ) ;
#9100=FACE_OUTER_BOUND ( 'NONE', #123829, .T. ) ;
#9101=CIRCLE ( 'NONE', #82274, 0.06509327318403745899 ) ;
#9102=ORIENTED_EDGE ( 'NONE', *, *, #19385, .F. ) ;
#9103=EDGE_CURVE ( 'NONE', #49010, #20499, #21410, .T. ) ;
#9104=ORIENTED_EDGE ( 'NONE', *, *, #68196, .T. ) ;
#9106=ADVANCED_FACE ( 'NONE', ( #2128 ), #20498, .T. ) ;
#9107=ORIENTED_EDGE ( 'NONE', *, *, #41940, .F. ) ;
#9108=CONICAL_SURFACE ( 'NONE', #32121, 0.1000000000000002554, 0.003490658503988666988 ) ;
#9109=DIRECTION ( 'NONE',  ( 0.000000000000000000, 0.000000000000000000, 1.000000000000000000 ) ) ;
#9110=DIRECTION ( 'NONE',  ( 0.000000000000000000, 0.000000000000000000, 1.000000000000000000 ) ) ;
#9111=CONICAL_SURFACE ( 'NONE', #61457, 0.1000000000000000472, 0.003490658503988666988 ) ;
#9112=EDGE_CURVE ( 'NONE', #51138, #104697, #42069, .T. ) ;
#9113=CIRCLE ( 'NONE', #76010, 0.06509327318403745899 ) ;
#9114=ORIENTED_EDGE ( 'NONE', *, *, #41042, .T. ) ;
#9115=EDGE_CURVE ( 'NONE', #91937, #87854, #71588, .T. ) ;
#9116=LINE ( 'NONE', #41185, #98766 ) ;
#9117=AXIS2_PLACEMENT_3D ( 'NONE', #128773, #125035, #115859 ) ;
#9118=CARTESIAN_POINT ( 'NONE',  ( 17.50000000000000000, -2.750000000000000444, -2.864912725862979848 ) ) ;
#9119=EDGE_CURVE ( 'NONE', #70277, #85577, #119697, .T. ) ;
#9120=DIRECTION ( 'NONE',  ( -0.000000000000000000, 1.000000000000000000, -0.000000000000000000 ) ) ;
#9121=DIRECTION ( 'NONE',  ( 0.000000000000000000, 0.000000000000000000, 1.000000000000000000 ) ) ;
#9122=VERTEX_POINT ( 'NONE', #12588 ) ;
#9123=DIRECTION ( 'NONE',  ( -0.000000000000000000, 1.000000000000000000, -0.000000000000000000 ) ) ;
#9124=CIRCLE ( 'NONE', #11258, 0.1000000000000002554 ) ;
#9125=EDGE_CURVE ( 'NONE', #98405, #128034, #11309, .T. ) ;
#9126=CARTESIAN_POINT ( 'NONE',  ( 5.399999999999935518, 12.50000000000000000, -4.395220292106239768 ) ) ;
#9127=ORIENTED_EDGE ( 'NONE', *, *, #55767, .T. ) ;
#9128=CONICAL_SURFACE ( 'NONE', #34186, 0.1000000000000002554, 0.003490658503988666988 ) ;
#9129=AXIS2_PLACEMENT_3D ( 'NONE', #72224, #22490, #32317 ) ;
#9130=CIRCLE ( 'NONE', #17524, 0.06509327318403745899 ) ;
#9131=ORIENTED_EDGE ( 'NONE', *, *, #56503, .F. ) ;
#9132=VERTEX_POINT ( 'NONE', #19853 ) ;
#9133=VERTEX_POINT ( 'NONE', #112099 ) ;
#9134=CARTESIAN_POINT ( 'NONE',  ( 6.849999999999929479, 12.50000000000000000, -2.511473670974877948 ) ) ;
#9135=CONICAL_SURFACE ( 'NONE', #101072, 0.1000000000000002554, 0.003490658503988666988 ) ;
#9136=CARTESIAN_POINT ( 'NONE',  ( 13.34999999999989662, 2.500000000000000000, -2.857883832488653741 ) ) ;
#9137=AXIS2_PLACEMENT_3D ( 'NONE', #95143, #15916, #93217 ) ;
#9138=VERTEX_POINT ( 'NONE', #52522 ) ;
#9139=DIRECTION ( 'NONE',  ( -0.000000000000000000, -1.000000000000000000, -0.000000000000000000 ) ) ;
#9140=CARTESIAN_POINT ( 'NONE',  ( -2.900000000000029221, 12.50000000000000000, -4.330127018922201643 ) ) ;
#9141=DIRECTION ( 'NONE',  ( 0.000000000000000000, 0.000000000000000000, -1.000000000000000000 ) ) ;
#9142=DIRECTION ( 'NONE',  ( 0.000000000000000000, -0.9999939076577903929, 0.003490651415223739937 ) ) ;
#9143=EDGE_CURVE ( 'NONE', #51919, #71123, #10635, .T. ) ;
#9144=ORIENTED_EDGE ( 'NONE', *, *, #78306, .T. ) ;
#9145=CARTESIAN_POINT ( 'NONE',  ( 4.549999999999935874, 2.500000000000000000, 6.595190528383296780 ) ) ;
#9146=EDGE_LOOP ( 'NONE', ( #115940, #29496 ) ) ;
#9147=EDGE_LOOP ( 'NONE', ( #59259, #65933 ) ) ;
#9148=DIRECTION ( 'NONE',  ( -0.000000000000000000, 1.000000000000000000, -0.000000000000000000 ) ) ;
#9149=CONICAL_SURFACE ( 'NONE', #53071, 0.1000000000000002554, 0.003490658503988666988 ) ;
#9150=AXIS2_PLACEMENT_3D ( 'NONE', #14330, #54277, #94199 ) ;
#9151=CARTESIAN_POINT ( 'NONE',  ( 11.64999999999990443, 2.500000000000000000, 1.572243186433545548 ) ) ;
#9152=FACE_BOUND ( 'NONE', #53337, .T. ) ;
#9153=DIRECTION ( 'NONE',  ( 0.000000000000000000, 1.000000000000000000, 0.000000000000000000 ) ) ;
#9154=DIRECTION ( 'NONE',  ( 0.000000000000000000, 0.000000000000000000, -1.000000000000000000 ) ) ;
#9155=LINE ( 'NONE', #22224, #73195 ) ;
#9156=CIRCLE ( 'NONE', #90728, 0.1000000000000000472 ) ;
#9157=CIRCLE ( 'NONE', #82332, 0.06509327318403741736 ) ;
#9158=ADVANCED_FACE ( 'NONE', ( #30979 ), #44490, .T. ) ;
#9159=CIRCLE ( 'NONE', #28036, 0.09999999999999982514 ) ;
#9160=AXIS2_PLACEMENT_3D ( 'NONE', #29212, #67818, #88077 ) ;
#9161=ORIENTED_EDGE ( 'NONE', *, *, #22010, .F. ) ;
#9162=CARTESIAN_POINT ( 'NONE',  ( 4.349999999999940137, 2.500000000000000000, -2.611473670974877592 ) ) ;
#9163=DIRECTION ( 'NONE',  ( -0.000000000000000000, 1.000000000000000000, -0.000000000000000000 ) ) ;
#9164=DIRECTION ( 'NONE',  ( -0.000000000000000000, -1.000000000000000000, -0.000000000000000000 ) ) ;
#9165=DIRECTION ( 'NONE',  ( -0.000000000000000000, 1.000000000000000000, -0.000000000000000000 ) ) ;
#9166=ORIENTED_EDGE ( 'NONE', *, *, #102502, .F. ) ;
#9167=PLANE ( 'NONE',  #34374 ) ;
#9168=AXIS2_PLACEMENT_3D ( 'NONE', #63654, #103579, #44014 ) ;
#9169=VECTOR ( 'NONE', #26415, 1000.000000000000000 ) ;
#9170=DIRECTION ( 'NONE',  ( 0.000000000000000000, 1.000000000000000000, 0.000000000000000000 ) ) ;
#9171=ORIENTED_EDGE ( 'NONE', *, *, #89424, .T. ) ;
#9172=ORIENTED_EDGE ( 'NONE', *, *, #69173, .F. ) ;
#9173=AXIS2_PLACEMENT_3D ( 'NONE', #32143, #91038, #52400 ) ;
#9174=DIRECTION ( 'NONE',  ( -0.000000000000000000, -1.000000000000000000, -0.000000000000000000 ) ) ;
#9175=ADVANCED_FACE ( 'NONE', ( #11951 ), #80712, .T. ) ;
#9176=DIRECTION ( 'NONE',  ( 0.000000000000000000, 1.000000000000000000, 0.000000000000000000 ) ) ;
#9177=FACE_BOUND ( 'NONE', #25366, .T. ) ;
#9178=DIRECTION ( 'NONE',  ( 0.000000000000000000, 0.000000000000000000, 1.000000000000000000 ) ) ;
#9179=VERTEX_POINT ( 'NONE', #121268 ) ;
#9180=CARTESIAN_POINT ( 'NONE',  ( -12.29999999999999538, 2.500000000000000000, 4.676537180435972552 ) ) ;
#9181=VERTEX_POINT ( 'NONE', #70240 ) ;
#9182=LINE ( 'NONE', #47183, #105103 ) ;
#9184=CIRCLE ( 'NONE', #119907, 0.06509327318403745899 ) ;
#9185=ORIENTED_EDGE ( 'NONE', *, *, #102178, .T. ) ;
#9186=CARTESIAN_POINT ( 'NONE',  ( 5.849999999999933920, 2.500000000000000000, -2.165063509461101710 ) ) ;
#9187=DIRECTION ( 'NONE',  ( 0.000000000000000000, 0.000000000000000000, 1.000000000000000000 ) ) ;
#9188=DIRECTION ( 'NONE',  ( 0.000000000000000000, 0.000000000000000000, 1.000000000000000000 ) ) ;
#9189=CARTESIAN_POINT ( 'NONE',  ( -12.89999999999999325, 12.50000000000000000, 0.6928203230275535862 ) ) ;
#9190=VECTOR ( 'NONE', #65523, 1000.000000000000000 ) ;
#9191=AXIS2_PLACEMENT_3D ( 'NONE', #84506, #124431, #34776 ) ;
#9192=ORIENTED_EDGE ( 'NONE', *, *, #18573, .T. ) ;
#9193=ADVANCED_FACE ( 'NONE', ( #31604 ), #6807, .T. ) ;
#9194=DIRECTION ( 'NONE',  ( 0.000000000000000000, 1.000000000000000000, 0.000000000000000000 ) ) ;
#9195=DIRECTION ( 'NONE',  ( 0.000000000000000000, -0.9999939076577903929, 0.003490651415223739937 ) ) ;
#9196=LINE ( 'NONE', #49146, #36762 ) ;
#9197=DIRECTION ( 'NONE',  ( 0.000000000000000000, 1.000000000000000000, 0.000000000000000000 ) ) ;
#9198=ORIENTED_EDGE ( 'NONE', *, *, #21995, .T. ) ;
#9199=ORIENTED_EDGE ( 'NONE', *, *, #115736, .F. ) ;
#9200=CARTESIAN_POINT ( 'NONE',  ( 16.56576425165006938, 2.500000000000000000, 6.084390597445819893 ) ) ;
#9201=ORIENTED_EDGE ( 'NONE', *, *, #50891, .T. ) ;
#9202=AXIS2_PLACEMENT_3D ( 'NONE', #114817, #104992, #94538 ) ;
#9203=PLANE ( 'NONE',  #84832 ) ;
#9204=DIRECTION ( 'NONE',  ( -0.000000000000000000, 1.000000000000000000, -0.000000000000000000 ) ) ;
#9205=CONICAL_SURFACE ( 'NONE', #40538, 0.09999999999999982514, 0.003490658503988666988 ) ;
#9206=DIRECTION ( 'NONE',  ( -0.000000000000000000, -1.000000000000000000, -0.000000000000000000 ) ) ;
#9207=DIRECTION ( 'NONE',  ( 0.000000000000000000, 0.000000000000000000, 1.000000000000000000 ) ) ;
#9208=ORIENTED_EDGE ( 'NONE', *, *, #114771, .F. ) ;
#9209=CARTESIAN_POINT ( 'NONE',  ( 7.899999999999924860, 2.500000000000000000, 4.430127018922196847 ) ) ;
#9210=FACE_OUTER_BOUND ( 'NONE', #663, .T. ) ;
#9211=CARTESIAN_POINT ( 'NONE',  ( 81.97620162060584903, 3.937821635701168166, -6.124242818032728408 ) ) ;
#9212=EDGE_CURVE ( 'NONE', #92207, #61030, #184, .T. ) ;
#9213=EDGE_CURVE ( 'NONE', #40443, #106006, #79993, .T. ) ;
#9214=CARTESIAN_POINT ( 'NONE',  ( 13.34999999999989662, 2.500000000000000000, -2.165063509461101710 ) ) ;
#9215=PLANE ( 'NONE',  #105069 ) ;
#9216=EDGE_CURVE ( 'NONE', #126539, #108133, #125959, .T. ) ;
#9217=EDGE_CURVE ( 'NONE', #65457, #113749, #80056, .T. ) ;
#9218=CARTESIAN_POINT ( 'NONE',  ( -14.54999999999998472, 2.500000000000000000, 2.065063509461101621 ) ) ;
#9219=ORIENTED_EDGE ( 'NONE', *, *, #120553, .T. ) ;
#9220=ORIENTED_EDGE ( 'NONE', *, *, #28587, .F. ) ;
#9221=DIRECTION ( 'NONE',  ( 0.000000000000000000, 1.000000000000000000, 0.000000000000000000 ) ) ;
#9222=CIRCLE ( 'NONE', #126203, 0.06509327318403745899 ) ;
#9223=EDGE_LOOP ( 'NONE', ( #78376, #128382 ) ) ;
#9224=CONICAL_SURFACE ( 'NONE', #36430, 0.1000000000000002554, 0.003490658503988666988 ) ;
#9225=VECTOR ( 'NONE', #42677, 1000.000000000000000 ) ;
#9227=ORIENTED_EDGE ( 'NONE', *, *, #129400, .T. ) ;
#9228=ORIENTED_EDGE ( 'NONE', *, *, #62204, .T. ) ;
#9229=EDGE_LOOP ( 'NONE', ( #110914, #111984, #58646, #110071 ) ) ;
#9230=AXIS2_PLACEMENT_3D ( 'NONE', #94501, #44125, #6739 ) ;
#9231=EDGE_CURVE ( 'NONE', #83779, #129184, #84189, .T. ) ;
#9232=LINE ( 'NONE', #48510, #112762 ) ;
#9233=AXIS2_PLACEMENT_3D ( 'NONE', #120885, #42335, #121514 ) ;
#9234=ADVANCED_FACE ( 'NONE', ( #50584 ), #62363, .T. ) ;
#9235=CARTESIAN_POINT ( 'NONE',  ( 11.64999999999990266, 2.500000000000000000, -6.495190528383302464 ) ) ;
#9236=EDGE_CURVE ( 'NONE', #75526, #26170, #96704, .T. ) ;
#9237=PLANE ( 'NONE',  #24690 ) ;
#9239=DIRECTION ( 'NONE',  ( -0.000000000000000000, -1.000000000000000000, -0.000000000000000000 ) ) ;
#9240=DIRECTION ( 'NONE',  ( -0.000000000000000000, 1.000000000000000000, -0.000000000000000000 ) ) ;
#9241=DIRECTION ( 'NONE',  ( 0.000000000000000000, 1.000000000000000000, 0.000000000000000000 ) ) ;
#9242=CARTESIAN_POINT ( 'NONE',  ( 5.649999999999934630, 12.50000000000000000, 6.841600689897072485 ) ) ;
#9243=CARTESIAN_POINT ( 'NONE',  ( 0.8499999999999536815, 2.500000000000000000, 5.802370205355744659 ) ) ;
#9244=ORIENTED_EDGE ( 'NONE', *, *, #34204, .T. ) ;
#9245=ORIENTED_EDGE ( 'NONE', *, *, #90779, .F. ) ;
#9246=CONICAL_SURFACE ( 'NONE', #15486, 0.09999999999999982514, 0.003490658503988666988 ) ;
#9247=DIRECTION ( 'NONE',  ( -0.000000000000000000, -1.000000000000000000, -0.000000000000000000 ) ) ;
#9248=CONICAL_SURFACE ( 'NONE', #97067, 0.09999999999999982514, 0.003490658503988666988 ) ;
#9249=CIRCLE ( 'NONE', #86594, 0.06509327318403743123 ) ;
#9250=ORIENTED_EDGE ( 'NONE', *, *, #648, .T. ) ;
#9251=EDGE_LOOP ( 'NONE', ( #45064, #72272, #77640, #4723 ) ) ;
#9252=FACE_OUTER_BOUND ( 'NONE', #89003, .T. ) ;
#9253=AXIS2_PLACEMENT_3D ( 'NONE', #18482, #7364, #57778 ) ;
#9254=CIRCLE ( 'NONE', #25986, 0.1000000000000002554 ) ;
#9255=DIRECTION ( 'NONE',  ( -0.000000000000000000, 1.000000000000000000, -0.000000000000000000 ) ) ;
#9256=VECTOR ( 'NONE', #25708, 1000.000000000000000 ) ;
#9257=FACE_OUTER_BOUND ( 'NONE', #52603, .T. ) ;
#9258=DIRECTION ( 'NONE',  ( -0.000000000000000000, 1.000000000000000000, -0.000000000000000000 ) ) ;
#9259=LINE ( 'NONE', #12467, #124001 ) ;
#9260=ORIENTED_EDGE ( 'NONE', *, *, #87253, .F. ) ;
#9261=CIRCLE ( 'NONE', #19419, 0.06509327318403745899 ) ;
#9262=AXIS2_PLACEMENT_3D ( 'NONE', #47102, #49687, #108584 ) ;
#9263=ORIENTED_EDGE ( 'NONE', *, *, #74711, .T. ) ;
#9264=CARTESIAN_POINT ( 'NONE',  ( 10.39999999999991154, 2.500000000000000000, -3.637306695894650055 ) ) ;
#9265=CONICAL_SURFACE ( 'NONE', #76163, 0.09999999999999999167, 0.003490658503988666988 ) ;
#9266=ORIENTED_EDGE ( 'NONE', *, *, #42339, .T. ) ;
#9267=CARTESIAN_POINT ( 'NONE',  ( -9.800000000000004263, 2.500000000000000000, -0.4464101615137783252 ) ) ;
#9269=CIRCLE ( 'NONE', #92908, 0.06509327318403745899 ) ;
#9270=ORIENTED_EDGE ( 'NONE', *, *, #47643, .T. ) ;
#9271=LINE ( 'NONE', #97646, #94227 ) ;
#9272=FACE_OUTER_BOUND ( 'NONE', #71385, .T. ) ;
#9273=EDGE_CURVE ( 'NONE', #113704, #117157, #121847, .T. ) ;
#9274=DIRECTION ( 'NONE',  ( 0.000000000000000000, 0.000000000000000000, 1.000000000000000000 ) ) ;
#9275=DIRECTION ( 'NONE',  ( 0.000000000000000000, 0.000000000000000000, -1.000000000000000000 ) ) ;
#9276=EDGE_CURVE ( 'NONE', #3365, #21424, #35943, .T. ) ;
#9277=DIRECTION ( 'NONE',  ( -0.000000000000000000, 1.000000000000000000, -0.000000000000000000 ) ) ;
#9279=FACE_OUTER_BOUND ( 'NONE', #19632, .T. ) ;
#9280=CARTESIAN_POINT ( 'NONE',  ( -11.89999999999999680, 2.500000000000000000, -4.576537180435975571 ) ) ;
#9281=CARTESIAN_POINT ( 'NONE',  ( -12.09999999999999609, 12.50000000000000000, -3.572213422710609709 ) ) ;
#9282=DIRECTION ( 'NONE',  ( 0.000000000000000000, 0.000000000000000000, 1.000000000000000000 ) ) ;
#9283=VECTOR ( 'NONE', #95610, 1000.000000000000000 ) ;
#9284=EDGE_CURVE ( 'NONE', #77431, #129270, #19346, .T. ) ;
#9285=CARTESIAN_POINT ( 'NONE',  ( 13.74999999999989342, 2.500000000000000000, -1.572243186433550211 ) ) ;
#9286=ORIENTED_EDGE ( 'NONE', *, *, #110864, .F. ) ;
#9287=ORIENTED_EDGE ( 'NONE', *, *, #30866, .F. ) ;
#9288=DIRECTION ( 'NONE',  ( -0.000000000000000000, 1.000000000000000000, -0.000000000000000000 ) ) ;
#9289=ORIENTED_EDGE ( 'NONE', *, *, #62439, .F. ) ;
#9290=AXIS2_PLACEMENT_3D ( 'NONE', #14164, #81627, #32563 ) ;
#9291=CARTESIAN_POINT ( 'NONE',  ( 10.44999999999991402, 2.500000000000000000, 6.395190528383296602 ) ) ;
#9292=LINE ( 'NONE', #89138, #81632 ) ;
#9293=VECTOR ( 'NONE', #23489, 1000.000000000000000 ) ;
#9294=EDGE_LOOP ( 'NONE', ( #61885, #121794, #22820, #124223 ) ) ;
#9295=DIRECTION ( 'NONE',  ( 0.000000000000000000, 0.000000000000000000, -1.000000000000000000 ) ) ;
#9296=CARTESIAN_POINT ( 'NONE',  ( -13.74999999999998757, 12.50000000000000000, -2.922977105672689202 ) ) ;
#9297=LINE ( 'NONE', #70159, #79625 ) ;
#9298=CARTESIAN_POINT ( 'NONE',  ( 7.499999999999961808, 2.500000000000000000, -4.230127018922201998 ) ) ;
#9299=ORIENTED_EDGE ( 'NONE', *, *, #54776, .F. ) ;
#9300=CONICAL_SURFACE ( 'NONE', #40630, 0.1000000000000002554, 0.003490658503988666988 ) ;
#9301=CARTESIAN_POINT ( 'NONE',  ( 6.249999999999967137, 12.50000000000000000, 6.430097255199259010 ) ) ;
#9302=ORIENTED_EDGE ( 'NONE', *, *, #14775, .T. ) ;
#9303=DIRECTION ( 'NONE',  ( 0.000000000000000000, -0.000000000000000000, 1.000000000000000000 ) ) ;
#9304=DIRECTION ( 'NONE',  ( -0.000000000000000000, -1.000000000000000000, -0.000000000000000000 ) ) ;
#9305=CARTESIAN_POINT ( 'NONE',  ( -0.8500000000000382805, 12.50000000000000000, -7.253104124594891289 ) ) ;
#9306=ORIENTED_EDGE ( 'NONE', *, *, #97306, .T. ) ;
#9307=AXIS2_PLACEMENT_3D ( 'NONE', #52457, #779, #70812 ) ;
#9308=VECTOR ( 'NONE', #32852, 1000.000000000000000 ) ;
#9309=DIRECTION ( 'NONE',  ( -4.274815082592931898E-19, -0.9999939076577903929, -0.003490651415223739937 ) ) ;
#9310=EDGE_CURVE ( 'NONE', #128257, #26935, #40304, .T. ) ;
#9311=AXIS2_PLACEMENT_3D ( 'NONE', #100320, #41414, #61696 ) ;
#9312=ORIENTED_EDGE ( 'NONE', *, *, #54705, .F. ) ;
#9313=CARTESIAN_POINT ( 'NONE',  ( -5.850000000000022737, 2.500000000000000000, -2.265063509461101798 ) ) ;
#9314=CARTESIAN_POINT ( 'NONE',  ( -5.800000000000018474, 2.500000000000000000, 4.330127018922196314 ) ) ;
#9315=CARTESIAN_POINT ( 'NONE',  ( -2.050000000000033129, 12.50000000000000000, 2.165063509461097713 ) ) ;
#9316=EDGE_LOOP ( 'NONE', ( #44407, #107328, #14188, #28135 ) ) ;
#9317=CARTESIAN_POINT ( 'NONE',  ( 10.79999999999991012, 2.500000000000000000, -4.230127018922201998 ) ) ;
#9318=CARTESIAN_POINT ( 'NONE',  ( -12.49999999999999467, 2.500000000000000000, -3.737306695894647035 ) ) ;
#9319=ADVANCED_FACE ( 'NONE', ( #106608 ), #113444, .T. ) ;
#9320=ORIENTED_EDGE ( 'NONE', *, *, #121331, .F. ) ;
#9321=CARTESIAN_POINT ( 'NONE',  ( -11.25000000000000178, 2.500000000000000000, -5.802370205355746435 ) ) ;
#9322=ADVANCED_FACE ( 'NONE', ( #16279 ), #66042, .T. ) ;
#9323=ORIENTED_EDGE ( 'NONE', *, *, #60627, .F. ) ;
#9324=CARTESIAN_POINT ( 'NONE',  ( -13.14999999999999147, 12.50000000000000000, 1.818653347947325472 ) ) ;
#9325=CIRCLE ( 'NONE', #67907, 0.1000000000000002554 ) ;
#9326=ORIENTED_EDGE ( 'NONE', *, *, #50753, .T. ) ;
#9327=DIRECTION ( 'NONE',  ( 0.000000000000000000, 1.000000000000000000, 0.000000000000000000 ) ) ;
#9328=CARTESIAN_POINT ( 'NONE',  ( -5.000000000000026645, 12.50000000000000000, -3.637306695894650055 ) ) ;
#9329=VECTOR ( 'NONE', #78992, 1000.000000000000000 ) ;
#9330=CONICAL_SURFACE ( 'NONE', #3085, 0.1000000000000000056, 0.003490658503988666988 ) ;
#9331=ORIENTED_EDGE ( 'NONE', *, *, #20867, .T. ) ;
#9332=ADVANCED_FACE ( 'NONE', ( #47064 ), #25599, .T. ) ;
#9333=ORIENTED_EDGE ( 'NONE', *, *, #124504, .F. ) ;
#9334=LINE ( 'NONE', #6722, #117774 ) ;
#9335=DIRECTION ( 'NONE',  ( 0.000000000000000000, 0.000000000000000000, 1.000000000000000000 ) ) ;
#9336=ORIENTED_EDGE ( 'NONE', *, *, #112503, .T. ) ;
#9337=PLANE ( 'NONE',  #92809 ) ;
#9339=AXIS2_PLACEMENT_3D ( 'NONE', #122908, #82992, #24061 ) ;
#9340=CIRCLE ( 'NONE', #26077, 0.06509327318403741736 ) ;
#9341=VECTOR ( 'NONE', #44721, 1000.000000000000000 ) ;
#9342=CARTESIAN_POINT ( 'NONE',  ( -1.650000000000035216, 2.500000000000000000, -5.902370205355750521 ) ) ;
#9344=LINE ( 'NONE', #97081, #53027 ) ;
#9345=AXIS2_PLACEMENT_3D ( 'NONE', #69310, #109239, #100085 ) ;
#9347=CARTESIAN_POINT ( 'NONE',  ( 10.64999999999991331, 2.500000000000000000, 6.841600689897072485 ) ) ;
#9348=CIRCLE ( 'NONE', #1034, 0.1000000000000002554 ) ;
#9349=CIRCLE ( 'NONE', #7186, 0.06509327318403745899 ) ;
#9350=ORIENTED_EDGE ( 'NONE', *, *, #19285, .T. ) ;
#9351=EDGE_CURVE ( 'NONE', #9179, #91328, #63647, .T. ) ;
#9352=ORIENTED_EDGE ( 'NONE', *, *, #83133, .F. ) ;
#9353=VERTEX_POINT ( 'NONE', #97434 ) ;
#9354=EDGE_LOOP ( 'NONE', ( #46928, #53020 ) ) ;
#9355=DIRECTION ( 'NONE',  ( 0.000000000000000000, 0.000000000000000000, -1.000000000000000000 ) ) ;
#9356=DIRECTION ( 'NONE',  ( 0.000000000000000000, 0.000000000000000000, 1.000000000000000000 ) ) ;
#9357=VECTOR ( 'NONE', #115014, 1000.000000000000000 ) ;
#9358=FACE_OUTER_BOUND ( 'NONE', #106855, .T. ) ;
#9359=ORIENTED_EDGE ( 'NONE', *, *, #102783, .F. ) ;
#9360=FACE_BOUND ( 'NONE', #125009, .T. ) ;
#9361=ORIENTED_EDGE ( 'NONE', *, *, #47864, .F. ) ;
#9362=DIRECTION ( 'NONE',  ( 0.000000000000000000, 1.000000000000000000, 0.000000000000000000 ) ) ;
#9363=CARTESIAN_POINT ( 'NONE',  ( -12.29999999999999538, 12.50000000000000000, -0.3464101615137741841 ) ) ;
#9364=CARTESIAN_POINT ( 'NONE',  ( -11.64999999999999680, 2.500000000000000000, -2.265063509461097802 ) ) ;
#9365=ADVANCED_FACE ( 'NONE', ( #102903 ), #100909, .T. ) ;
#9366=DIRECTION ( 'NONE',  ( 0.000000000000000000, -0.9999939076577903929, 0.003490651415223739937 ) ) ;
#9367=DIRECTION ( 'NONE',  ( -0.000000000000000000, 1.000000000000000000, -0.000000000000000000 ) ) ;
#9368=CARTESIAN_POINT ( 'NONE',  ( -7.700000000000010836, 2.500000000000000000, 4.083716857408421497 ) ) ;
#9369=FACE_OUTER_BOUND ( 'NONE', #29517, .T. ) ;
#9370=CARTESIAN_POINT ( 'NONE',  ( 13.74999999999989519, 12.50000000000000000, -2.857883832488653741 ) ) ;
#9371=EDGE_CURVE ( 'NONE', #103567, #60985, #33548, .T. ) ;
#9372=ADVANCED_FACE ( 'NONE', ( #17577 ), #564, .T. ) ;
#9373=LINE ( 'NONE', #89219, #47405 ) ;
#9374=EDGE_CURVE ( 'NONE', #10577, #125752, #50761, .T. ) ;
#9375=EDGE_CURVE ( 'NONE', #63575, #41663, #32910, .T. ) ;
#9376=AXIS2_PLACEMENT_3D ( 'NONE', #85876, #125181, #125799 ) ;
#9377=CARTESIAN_POINT ( 'NONE',  ( -0.8500000000000390576, 12.50000000000000000, -2.165063509461101710 ) ) ;
#9378=ORIENTED_EDGE ( 'NONE', *, *, #76459, .T. ) ;
#9379=EDGE_LOOP ( 'NONE', ( #89695, #43189, #92876, #122815 ) ) ;
#9380=ORIENTED_EDGE ( 'NONE', *, *, #111507, .F. ) ;
#9381=ORIENTED_EDGE ( 'NONE', *, *, #74890, .T. ) ;
#9382=CARTESIAN_POINT ( 'NONE',  ( 17.45053073489777873, -1.969617801096962495, -4.507369966543559592 ) ) ;
#9383=EDGE_CURVE ( 'NONE', #30984, #91594, #65414, .T. ) ;
#9384=DIRECTION ( 'NONE',  ( 0.000000000000000000, 0.000000000000000000, -1.000000000000000000 ) ) ;
#9385=EDGE_CURVE ( 'NONE', #100404, #15576, #69521, .T. ) ;
#9386=EDGE_LOOP ( 'NONE', ( #18804, #64629 ) ) ;
#9387=ORIENTED_EDGE ( 'NONE', *, *, #57398, .F. ) ;
#9388=EDGE_LOOP ( 'NONE', ( #75653, #25072, #100050, #31211 ) ) ;
#9390=AXIS2_PLACEMENT_3D ( 'NONE', #122699, #33053, #63130 ) ;
#9391=CONICAL_SURFACE ( 'NONE', #76281, 0.1000000000000002554, 0.003490658503988666988 ) ;
#9392=EDGE_CURVE ( 'NONE', #2451, #10395, #65310, .T. ) ;
#9393=ADVANCED_FACE ( 'NONE', ( #72820 ), #123901, .T. ) ;
#9394=CARTESIAN_POINT ( 'NONE',  ( -9.150000000000009237, 2.500000000000000000, -1.372243186433550033 ) ) ;
#9395=DIRECTION ( 'NONE',  ( 0.000000000000000000, 0.000000000000000000, -1.000000000000000000 ) ) ;
#9396=DIRECTION ( 'NONE',  ( -0.000000000000000000, 1.000000000000000000, -0.000000000000000000 ) ) ;
#9397=DIRECTION ( 'NONE',  ( 0.000000000000000000, 0.000000000000000000, -1.000000000000000000 ) ) ;
#9398=CARTESIAN_POINT ( 'NONE',  ( 14.99999999999992895, 2.500000000000000000, 0.09999999999999772959 ) ) ;
#9399=CARTESIAN_POINT ( 'NONE',  ( -3.550000000000027356, 2.500000000000000000, -2.411473670974877859 ) ) ;
#9400=EDGE_LOOP ( 'NONE', ( #28922, #83238, #119882, #65804 ) ) ;
#9401=EDGE_CURVE ( 'NONE', #107047, #46462, #3423, .T. ) ;
#9402=CARTESIAN_POINT ( 'NONE',  ( 11.69999999999990870, 2.500000000000000000, 4.430127018922196847 ) ) ;
#9403=ORIENTED_EDGE ( 'NONE', *, *, #16123, .F. ) ;
#9404=CONICAL_SURFACE ( 'NONE', #53321, 0.1000000000000002554, 0.003490658503988666988 ) ;
#9405=ORIENTED_EDGE ( 'NONE', *, *, #79554, .T. ) ;
#9406=VERTEX_POINT ( 'NONE', #20170 ) ;
#9407=AXIS2_PLACEMENT_3D ( 'NONE', #26106, #46366, #26741 ) ;
#9408=DIRECTION ( 'NONE',  ( 0.000000000000000000, 1.000000000000000000, 0.000000000000000000 ) ) ;
#9409=VERTEX_POINT ( 'NONE', #128866 ) ;
#9410=VERTEX_POINT ( 'NONE', #18871 ) ;
#9411=DIRECTION ( 'NONE',  ( -4.274815082592931898E-19, -0.9999939076577903929, -0.003490651415223739937 ) ) ;
#9412=DIRECTION ( 'NONE',  ( 0.000000000000000000, 0.000000000000000000, 1.000000000000000000 ) ) ;
#9413=CARTESIAN_POINT ( 'NONE',  ( 2.099999999999950351, 2.500000000000000000, -0.6928203230275541413 ) ) ;
#9414=CONICAL_SURFACE ( 'NONE', #84627, 0.1000000000000002554, 0.003490658503988666988 ) ;
#9415=DIRECTION ( 'NONE',  ( 0.000000000000000000, 1.000000000000000000, 0.000000000000000000 ) ) ;
#9416=DIRECTION ( 'NONE',  ( 0.000000000000000000, 0.000000000000000000, 1.000000000000000000 ) ) ;
#9417=EDGE_LOOP ( 'NONE', ( #9018, #124719 ) ) ;
#9418=DIRECTION ( 'NONE',  ( 0.000000000000000000, 1.000000000000000000, 0.000000000000000000 ) ) ;
#9419=ORIENTED_EDGE ( 'NONE', *, *, #26086, .T. ) ;
#9420=CARTESIAN_POINT ( 'NONE',  ( 16.55712575656009733, 0.2764121571832068303, 6.093697237269479317 ) ) ;
#9421=VERTEX_POINT ( 'NONE', #58182 ) ;
#9423=CARTESIAN_POINT ( 'NONE',  ( -10.45000000000000462, 2.500000000000000000, -6.495190528383298911 ) ) ;
#9424=ORIENTED_EDGE ( 'NONE', *, *, #86245, .F. ) ;
#9425=DIRECTION ( 'NONE',  ( -0.000000000000000000, 1.000000000000000000, -0.000000000000000000 ) ) ;
#9426=CARTESIAN_POINT ( 'NONE',  ( 12.29999999999990123, 12.50000000000000000, 0.2813168883297361700 ) ) ;
#9427=CIRCLE ( 'NONE', #90984, 0.1000000000000002554 ) ;
#9428=VERTEX_POINT ( 'NONE', #58811 ) ;
#9430=AXIS2_PLACEMENT_3D ( 'NONE', #69729, #111586, #10774 ) ;
#9431=AXIS2_PLACEMENT_3D ( 'NONE', #17288, #76890, #14719 ) ;
#9432=CARTESIAN_POINT ( 'NONE',  ( 9.349999999999919709, 2.500000000000000000, 1.918653347947321564 ) ) ;
#9434=ORIENTED_EDGE ( 'NONE', *, *, #49696, .F. ) ;
#9435=VECTOR ( 'NONE', #34842, 1000.000000000000000 ) ;
#9436=ORIENTED_EDGE ( 'NONE', *, *, #8937, .F. ) ;
#9437=DIRECTION ( 'NONE',  ( -0.000000000000000000, 1.000000000000000000, -0.000000000000000000 ) ) ;
#9438=DIRECTION ( 'NONE',  ( -0.000000000000000000, 1.000000000000000000, -0.000000000000000000 ) ) ;
#9439=DIRECTION ( 'NONE',  ( 0.000000000000000000, 1.000000000000000000, 0.000000000000000000 ) ) ;
#9440=DIRECTION ( 'NONE',  ( 0.000000000000000000, 1.000000000000000000, 0.000000000000000000 ) ) ;
#9441=CIRCLE ( 'NONE', #40761, 0.1000000000000002554 ) ;
#9442=CARTESIAN_POINT ( 'NONE',  ( 9.599999999999917932, 2.500000000000000000, 0.6928203230275494784 ) ) ;
#9443=AXIS2_PLACEMENT_3D ( 'NONE', #123036, #90986, #1311 ) ;
#9444=ORIENTED_EDGE ( 'NONE', *, *, #44376, .F. ) ;
#9445=AXIS2_PLACEMENT_3D ( 'NONE', #108252, #99739, #27123 ) ;
#9446=DIRECTION ( 'NONE',  ( 0.000000000000000000, 0.000000000000000000, -1.000000000000000000 ) ) ;
#9448=ORIENTED_EDGE ( 'NONE', *, *, #34066, .F. ) ;
#9450=CARTESIAN_POINT ( 'NONE',  ( -4.400000000000025224, 12.50000000000000000, -0.3464101615137783474 ) ) ;
#9451=DIRECTION ( 'NONE',  ( 0.000000000000000000, 0.000000000000000000, 1.000000000000000000 ) ) ;
#9452=CONICAL_SURFACE ( 'NONE', #24030, 0.1000000000000000472, 0.003490658503988666988 ) ;
#9453=AXIS2_PLACEMENT_3D ( 'NONE', #80919, #61280, #88797 ) ;
#9454=CARTESIAN_POINT ( 'NONE',  ( 11.84999999999990727, 2.500000000000000000, -1.818653347947326138 ) ) ;
#9455=CARTESIAN_POINT ( 'NONE',  ( -1.050000000000037348, 12.50000000000000000, -2.446380397790840266 ) ) ;
#9456=DIRECTION ( 'NONE',  ( -4.274815082592931898E-19, -0.9999939076577903929, -0.003490651415223739937 ) ) ;
#9457=DIRECTION ( 'NONE',  ( 0.000000000000000000, 0.000000000000000000, 1.000000000000000000 ) ) ;
#9458=CARTESIAN_POINT ( 'NONE',  ( -4.550000000000026468, 12.50000000000000000, -6.495190528383302464 ) ) ;
#9459=ORIENTED_EDGE ( 'NONE', *, *, #74083, .T. ) ;
#9460=DIRECTION ( 'NONE',  ( 0.000000000000000000, 0.000000000000000000, 1.000000000000000000 ) ) ;
#9461=CARTESIAN_POINT ( 'NONE',  ( -11.05000000000000071, 12.50000000000000000, 6.776507416713035248 ) ) ;
#9463=CIRCLE ( 'NONE', #51254, 0.06509327318403745899 ) ;
#9464=ORIENTED_EDGE ( 'NONE', *, *, #122283, .T. ) ;
#9465=CARTESIAN_POINT ( 'NONE',  ( -11.25000000000000000, 2.500000000000000000, -7.088010851410849966 ) ) ;
#9466=EDGE_CURVE ( 'NONE', #106163, #34203, #109846, .T. ) ;
#9467=ORIENTED_EDGE ( 'NONE', *, *, #78260, .T. ) ;
#9468=VERTEX_POINT ( 'NONE', #59484 ) ;
#9469=FACE_OUTER_BOUND ( 'NONE', #125015, .T. ) ;
#9470=AXIS2_PLACEMENT_3D ( 'NONE', #51873, #121249, #23050 ) ;
#9471=ORIENTED_EDGE ( 'NONE', *, *, #62734, .T. ) ;
#9472=DIRECTION ( 'NONE',  ( -0.000000000000000000, -1.000000000000000000, -0.000000000000000000 ) ) ;
#9473=DIRECTION ( 'NONE',  ( 0.000000000000000000, 1.000000000000000000, 0.000000000000000000 ) ) ;
#9474=VECTOR ( 'NONE', #22593, 1000.000000000000000 ) ;
#9475=AXIS2_PLACEMENT_3D ( 'NONE', #62636, #82917, #50871 ) ;
#9476=VERTEX_POINT ( 'NONE', #88916 ) ;
#9477=DIRECTION ( 'NONE',  ( -4.274815082592931898E-19, -0.9999939076577903929, -0.003490651415223739937 ) ) ;
#9478=CARTESIAN_POINT ( 'NONE',  ( -4.400000000000025224, 2.500000000000000000, -0.3464101615137783474 ) ) ;
#9479=ORIENTED_EDGE ( 'NONE', *, *, #25895, .T. ) ;
#9480=EDGE_CURVE ( 'NONE', #85840, #17226, #82044, .T. ) ;
#9481=DIRECTION ( 'NONE',  ( 0.000000000000000000, 0.000000000000000000, 1.000000000000000000 ) ) ;
#9482=DIRECTION ( 'NONE',  ( -0.000000000000000000, -1.000000000000000000, -0.000000000000000000 ) ) ;
#9483=EDGE_CURVE ( 'NONE', #17558, #94655, #80100, .T. ) ;
#9484=ORIENTED_EDGE ( 'NONE', *, *, #98562, .T. ) ;
#9485=CIRCLE ( 'NONE', #63783, 0.06509327318403745899 ) ;
#9486=VERTEX_POINT ( 'NONE', #118363 ) ;
#9487=AXIS2_PLACEMENT_3D ( 'NONE', #98053, #117666, #89526 ) ;
#9488=ORIENTED_EDGE ( 'NONE', *, *, #86360, .T. ) ;
#9489=DIRECTION ( 'NONE',  ( 0.000000000000000000, 0.000000000000000000, 1.000000000000000000 ) ) ;
#9490=CARTESIAN_POINT ( 'NONE',  ( 2.899999999999944844, 2.500000000000000000, 3.637306695894644726 ) ) ;
#9491=CARTESIAN_POINT ( 'NONE',  ( -10.40000000000000213, 12.50000000000000000, -4.395220292106235327 ) ) ;
#9492=EDGE_CURVE ( 'NONE', #60798, #24108, #19438, .T. ) ;
#9493=FACE_BOUND ( 'NONE', #100702, .T. ) ;
#9494=VERTEX_POINT ( 'NONE', #28062 ) ;
#9495=CARTESIAN_POINT ( 'NONE',  ( 8.149999999999923972, 12.50000000000000000, -6.841600689897077814 ) ) ;
#9496=CARTESIAN_POINT ( 'NONE',  ( -4.350000000000027178, 2.500000000000000000, -6.148780366869526226 ) ) ;
#9497=ORIENTED_EDGE ( 'NONE', *, *, #61825, .F. ) ;
#9498=DIRECTION ( 'NONE',  ( -0.6795087154616692438, 6.363550617825454546E-16, -0.7336674352945157240 ) ) ;
#9499=AXIS2_PLACEMENT_3D ( 'NONE', #122036, #11426, #72926 ) ;
#9500=LINE ( 'NONE', #118801, #80523 ) ;
#9501=AXIS2_PLACEMENT_3D ( 'NONE', #831, #10624, #112732 ) ;
#9502=DIRECTION ( 'NONE',  ( -0.000000000000000000, -1.000000000000000000, -0.000000000000000000 ) ) ;
#9503=CARTESIAN_POINT ( 'NONE',  ( -9.550000000000006040, 2.500000000000000000, 2.165063509461097713 ) ) ;
#9504=DIRECTION ( 'NONE',  ( 0.000000000000000000, 1.000000000000000000, 0.000000000000000000 ) ) ;
#9505=DIRECTION ( 'NONE',  ( -0.000000000000000000, 1.000000000000000000, -0.000000000000000000 ) ) ;
#9506=DIRECTION ( 'NONE',  ( 0.000000000000000000, 0.000000000000000000, -1.000000000000000000 ) ) ;
#9507=VERTEX_POINT ( 'NONE', #99386 ) ;
#9508=ORIENTED_EDGE ( 'NONE', *, *, #43455, .F. ) ;
#9509=VERTEX_POINT ( 'NONE', #87610 ) ;
#9510=VECTOR ( 'NONE', #31929, 1000.000000000000000 ) ;
#9511=ORIENTED_EDGE ( 'NONE', *, *, #15275, .F. ) ;
#9512=ORIENTED_EDGE ( 'NONE', *, *, #119176, .T. ) ;
#9513=PLANE ( 'NONE',  #127940 ) ;
#9514=FACE_OUTER_BOUND ( 'NONE', #123325, .T. ) ;
#9515=VERTEX_POINT ( 'NONE', #60118 ) ;
#9516=FACE_BOUND ( 'NONE', #83588, .T. ) ;
#9517=VECTOR ( 'NONE', #100666, 1000.000000000000000 ) ;
#9518=DIRECTION ( 'NONE',  ( 0.000000000000000000, 1.000000000000000000, 0.000000000000000000 ) ) ;
#9519=EDGE_CURVE ( 'NONE', #57536, #117403, #9708, .T. ) ;
#9520=CONICAL_SURFACE ( 'NONE', #42904, 0.1000000000000002554, 0.003490658503988666988 ) ;
#9521=DIRECTION ( 'NONE',  ( 0.000000000000000000, 1.000000000000000000, 0.000000000000000000 ) ) ;
#9522=CIRCLE ( 'NONE', #28404, 0.1000000000000002554 ) ;
#9523=FACE_OUTER_BOUND ( 'NONE', #31925, .T. ) ;
#9524=DIRECTION ( 'NONE',  ( 0.000000000000000000, 0.000000000000000000, 1.000000000000000000 ) ) ;
#9525=FACE_OUTER_BOUND ( 'NONE', #112386, .T. ) ;
#9526=ADVANCED_FACE ( 'NONE', ( #69919 ), #42456, .T. ) ;
#9527=DIRECTION ( 'NONE',  ( 0.000000000000000000, 1.000000000000000000, 0.000000000000000000 ) ) ;
#9528=ORIENTED_EDGE ( 'NONE', *, *, #18097, .F. ) ;
#9529=ADVANCED_FACE ( 'NONE', ( #60744 ), #48803, .T. ) ;
#9530=AXIS2_PLACEMENT_3D ( 'NONE', #16474, #77993, #67503 ) ;
#9531=VERTEX_POINT ( 'NONE', #89553 ) ;
#9532=ORIENTED_EDGE ( 'NONE', *, *, #97864, .T. ) ;
#9533=EDGE_LOOP ( 'NONE', ( #14337, #32365 ) ) ;
#9534=ADVANCED_FACE ( 'NONE', ( #90173 ), #117722, .T. ) ;
#9535=CIRCLE ( 'NONE', #126516, 0.06509327318403745899 ) ;
#9536=CARTESIAN_POINT ( 'NONE',  ( 10.06913504599038589, 2.500000000000000444, 8.158951466667705432 ) ) ;
#9537=ADVANCED_FACE ( 'NONE', ( #80393 ), #101020, .T. ) ;
#9538=DIRECTION ( 'NONE',  ( 0.000000000000000000, -0.000000000000000000, 1.000000000000000000 ) ) ;
#9539=ADVANCED_FACE ( 'NONE', ( #49005 ), #39194, .T. ) ;
#9540=ORIENTED_EDGE ( 'NONE', *, *, #104981, .T. ) ;
#9541=DIRECTION ( 'NONE',  ( 0.000000000000000000, -0.000000000000000000, 1.000000000000000000 ) ) ;
#9542=VECTOR ( 'NONE', #80111, 1000.000000000000000 ) ;
#9543=AXIS2_PLACEMENT_3D ( 'NONE', #6748, #46711, #86627 ) ;
#9544=DIRECTION ( 'NONE',  ( 0.000000000000000000, 0.000000000000000000, 1.000000000000000000 ) ) ;
#9545=AXIS2_PLACEMENT_3D ( 'NONE', #19183, #101645, #29675 ) ;
#9546=DIRECTION ( 'NONE',  ( 0.000000000000000000, 0.000000000000000000, 1.000000000000000000 ) ) ;
#9547=EDGE_CURVE ( 'NONE', #4520, #78724, #25706, .T. ) ;
#9549=DIRECTION ( 'NONE',  ( -0.000000000000000000, -1.000000000000000000, -0.000000000000000000 ) ) ;
#9550=DIRECTION ( 'NONE',  ( 0.000000000000000000, 0.000000000000000000, 1.000000000000000000 ) ) ;
#9551=DIRECTION ( 'NONE',  ( 0.000000000000000000, 0.000000000000000000, 1.000000000000000000 ) ) ;
#9552=EDGE_LOOP ( 'NONE', ( #65835, #97726, #118168, #57625 ) ) ;
#9553=CARTESIAN_POINT ( 'NONE',  ( 7.499999999999961808, 12.50000000000000000, 4.265033745738159077 ) ) ;
#9554=EDGE_CURVE ( 'NONE', #72741, #106830, #98080, .T. ) ;
#9555=EDGE_LOOP ( 'NONE', ( #7857, #107446, #48874, #51348 ) ) ;
#9556=ORIENTED_EDGE ( 'NONE', *, *, #88559, .F. ) ;
#9557=DIRECTION ( 'NONE',  ( 0.000000000000000000, -0.000000000000000000, 1.000000000000000000 ) ) ;
#9558=CARTESIAN_POINT ( 'NONE',  ( -14.14999999999998614, 2.500000000000000000, -2.165063509461099489 ) ) ;
#9560=CIRCLE ( 'NONE', #53389, 0.06509327318403741736 ) ;
#9561=ORIENTED_EDGE ( 'NONE', *, *, #70626, .F. ) ;
#9562=EDGE_LOOP ( 'NONE', ( #126635, #7600 ) ) ;
#9563=CARTESIAN_POINT ( 'NONE',  ( 3.949999999999942446, 2.500000000000000000, -2.511473670974877948 ) ) ;
#9564=FACE_OUTER_BOUND ( 'NONE', #49629, .T. ) ;
#9565=CARTESIAN_POINT ( 'NONE',  ( 14.34999999999989306, 12.50000000000000000, -2.576566944158915184 ) ) ;
#9566=ORIENTED_EDGE ( 'NONE', *, *, #114056, .T. ) ;
#9567=DIRECTION ( 'NONE',  ( 0.000000000000000000, 1.000000000000000000, 0.000000000000000000 ) ) ;
#9568=AXIS2_PLACEMENT_3D ( 'NONE', #121725, #81794, #80533 ) ;
#9569=VECTOR ( 'NONE', #109503, 1000.000000000000000 ) ;
#9570=ORIENTED_EDGE ( 'NONE', *, *, #100064, .T. ) ;
#9571=CARTESIAN_POINT ( 'NONE',  ( 11.24999999999994316, 12.50000000000000000, 2.165063509461097713 ) ) ;
#9572=AXIS2_PLACEMENT_3D ( 'NONE', #70354, #42189, #21914 ) ;
#9573=EDGE_LOOP ( 'NONE', ( #16113, #91803 ) ) ;
#9574=AXIS2_PLACEMENT_3D ( 'NONE', #129129, #39463, #11898 ) ;
#9575=DIRECTION ( 'NONE',  ( -0.000000000000000000, 1.000000000000000000, -0.000000000000000000 ) ) ;
#9577=PLANE ( 'NONE',  #19715 ) ;
#9578=DIRECTION ( 'NONE',  ( 0.000000000000000000, -0.000000000000000000, 1.000000000000000000 ) ) ;
#9579=VERTEX_POINT ( 'NONE', #62687 ) ;
#9580=DIRECTION ( 'NONE',  ( -4.274815082592931898E-19, -0.9999939076577903929, -0.003490651415223739937 ) ) ;
#9581=EDGE_CURVE ( 'NONE', #125530, #102565, #96803, .T. ) ;
#9582=CONICAL_SURFACE ( 'NONE', #82754, 0.09999999999999982514, 0.003490658503988666988 ) ;
#9583=AXIS2_PLACEMENT_3D ( 'NONE', #100330, #86787, #27223 ) ;
#9584=ORIENTED_EDGE ( 'NONE', *, *, #108031, .F. ) ;
#9585=ORIENTED_EDGE ( 'NONE', *, *, #93523, .F. ) ;
#9586=FACE_OUTER_BOUND ( 'NONE', #20543, .T. ) ;
#9587=CARTESIAN_POINT ( 'NONE',  ( -5.850000000000018296, 12.50000000000000000, 7.253104124594885960 ) ) ;
#9588=CARTESIAN_POINT ( 'NONE',  ( -6.650000000000018119, 12.50000000000000000, -2.792790559304616504 ) ) ;
#9589=CARTESIAN_POINT ( 'NONE',  ( 12.09999999999990550, 12.50000000000000000, -4.330127018922201643 ) ) ;
#9590=CARTESIAN_POINT ( 'NONE',  ( -8.950000000000006395, 12.50000000000000000, 6.841600689897072485 ) ) ;
#9591=DIRECTION ( 'NONE',  ( -0.000000000000000000, -1.000000000000000000, -0.000000000000000000 ) ) ;
#9592=EDGE_CURVE ( 'NONE', #42850, #59613, #46640, .T. ) ;
#9593=CIRCLE ( 'NONE', #34655, 0.1000000000000002554 ) ;
#9594=CONICAL_SURFACE ( 'NONE', #30545, 0.1000000000000002554, 0.003490658503988666988 ) ;
#9595=DIRECTION ( 'NONE',  ( 0.000000000000000000, 0.000000000000000000, -1.000000000000000000 ) ) ;
#9596=CARTESIAN_POINT ( 'NONE',  ( -4.600000000000028955, 2.500000000000000000, -4.430127018922202176 ) ) ;
#9597=DIRECTION ( 'NONE',  ( 0.000000000000000000, -0.9999939076577903929, 0.003490651415223739937 ) ) ;
#9598=VERTEX_POINT ( 'NONE', #113711 ) ;
#9600=PLANE ( 'NONE',  #123148 ) ;
#9601=CARTESIAN_POINT ( 'NONE',  ( 0.6499999999999543920, 2.500000000000000000, 6.741600689897071952 ) ) ;
#9602=FACE_OUTER_BOUND ( 'NONE', #58722, .T. ) ;
#9603=DIRECTION ( 'NONE',  ( 0.000000000000000000, 0.000000000000000000, 1.000000000000000000 ) ) ;
#9604=ORIENTED_EDGE ( 'NONE', *, *, #84640, .F. ) ;
#9605=DIRECTION ( 'NONE',  ( -0.000000000000000000, -1.000000000000000000, -0.000000000000000000 ) ) ;
#9606=CIRCLE ( 'NONE', #40939, 0.06509327318403745899 ) ;
#9607=AXIS2_PLACEMENT_3D ( 'NONE', #20393, #11844, #110063 ) ;
#9608=CARTESIAN_POINT ( 'NONE',  ( 4.349999999999940137, 2.500000000000000000, -6.841600689897078702 ) ) ;
#9609=PLANE ( 'NONE',  #88055 ) ;
#9610=ORIENTED_EDGE ( 'NONE', *, *, #97126, .F. ) ;
#9611=ORIENTED_EDGE ( 'NONE', *, *, #44394, .T. ) ;
#9612=CONICAL_SURFACE ( 'NONE', #45418, 0.09999999999999982514, 0.003490658503988666988 ) ;
#9613=DIRECTION ( 'NONE',  ( -4.274815082592931898E-19, -0.9999939076577903929, -0.003490651415223739937 ) ) ;
#9614=ADVANCED_FACE ( 'NONE', ( #103248 ), #34130, .T. ) ;
#9615=EDGE_LOOP ( 'NONE', ( #94078, #21722, #26798, #60605 ) ) ;
#9616=ORIENTED_EDGE ( 'NONE', *, *, #35927, .T. ) ;
#9617=VERTEX_POINT ( 'NONE', #82967 ) ;
#9618=LINE ( 'NONE', #68533, #63357 ) ;
#9619=AXIS2_PLACEMENT_3D ( 'NONE', #106993, #56600, #66434 ) ;
#9620=DIRECTION ( 'NONE',  ( 0.000000000000000000, 0.000000000000000000, 1.000000000000000000 ) ) ;
#9621=DIRECTION ( 'NONE',  ( -4.274815082592931898E-19, -0.9999939076577903929, -0.003490651415223739937 ) ) ;
#9622=AXIS2_PLACEMENT_3D ( 'NONE', #116003, #26995, #66253 ) ;
#9623=LINE ( 'NONE', #8964, #20695 ) ;
#9624=EDGE_CURVE ( 'NONE', #95428, #62002, #23654, .T. ) ;
#9625=ORIENTED_EDGE ( 'NONE', *, *, #3190, .F. ) ;
#9626=CARTESIAN_POINT ( 'NONE',  ( -11.44999999999999929, 12.50000000000000000, -1.883746621131359600 ) ) ;
#9627=AXIS2_PLACEMENT_3D ( 'NONE', #92180, #101375, #50997 ) ;
#9628=ORIENTED_EDGE ( 'NONE', *, *, #72659, .F. ) ;
#9629=CARTESIAN_POINT ( 'NONE',  ( -13.74999999999995381, 12.50000000000000000, 2.165063509461101265 ) ) ;
#9630=EDGE_CURVE ( 'NONE', #27914, #66020, #109329, .T. ) ;
#9631=CARTESIAN_POINT ( 'NONE',  ( 18.93069778776535017, 2.571126379696623943, 2.451182541064385489 ) ) ;
#9632=CARTESIAN_POINT ( 'NONE',  ( 2.099999999999950351, 12.50000000000000000, -4.330127018922201643 ) ) ;
#9633=DIRECTION ( 'NONE',  ( -0.000000000000000000, 1.000000000000000000, -0.000000000000000000 ) ) ;
#9634=EDGE_CURVE ( 'NONE', #115142, #13760, #101956, .T. ) ;
#9635=EDGE_LOOP ( 'NONE', ( #112073, #54024 ) ) ;
#9636=EDGE_LOOP ( 'NONE', ( #33222, #99534 ) ) ;
#9637=EDGE_CURVE ( 'NONE', #67575, #106091, #63372, .T. ) ;
#9638=ORIENTED_EDGE ( 'NONE', *, *, #39541, .T. ) ;
#9639=EDGE_LOOP ( 'NONE', ( #68602, #26178 ) ) ;
#9640=ORIENTED_EDGE ( 'NONE', *, *, #3917, .T. ) ;
#9641=DIRECTION ( 'NONE',  ( 0.000000000000000000, 0.000000000000000000, 1.000000000000000000 ) ) ;
#9642=DIRECTION ( 'NONE',  ( -0.000000000000000000, -1.000000000000000000, -0.000000000000000000 ) ) ;
#9643=DIRECTION ( 'NONE',  ( 0.000000000000000000, 0.000000000000000000, -1.000000000000000000 ) ) ;
#9644=ADVANCED_FACE ( 'NONE', ( #123512 ), #51577, .T. ) ;
#9645=FACE_BOUND ( 'NONE', #23800, .T. ) ;
#9646=CARTESIAN_POINT ( 'NONE',  ( 1.049999999999952083, 12.50000000000000000, 6.906693963081109722 ) ) ;
#9647=CIRCLE ( 'NONE', #124576, 0.06509327318403745899 ) ;
#9648=DIRECTION ( 'NONE',  ( -0.000000000000000000, -1.000000000000000000, -0.000000000000000000 ) ) ;
#9649=CARTESIAN_POINT ( 'NONE',  ( 3.949999999999938893, 12.50000000000000000, 6.148780366869520009 ) ) ;
#9650=DIRECTION ( 'NONE',  ( 0.000000000000000000, 0.000000000000000000, 1.000000000000000000 ) ) ;
#9651=CIRCLE ( 'NONE', #43409, 0.1000000000000002554 ) ;
#9652=DIRECTION ( 'NONE',  ( 0.000000000000000000, 1.000000000000000000, 0.000000000000000000 ) ) ;
#9653=CIRCLE ( 'NONE', #41072, 0.06509327318403745899 ) ;
#9654=DIRECTION ( 'NONE',  ( 0.000000000000000000, 1.000000000000000000, 0.000000000000000000 ) ) ;
#9655=DIRECTION ( 'NONE',  ( 0.000000000000000000, -0.9999939076577903929, 0.003490651415223739937 ) ) ;
#9656=AXIS2_PLACEMENT_3D ( 'NONE', #66322, #47344, #54558 ) ;
#9657=CONICAL_SURFACE ( 'NONE', #103841, 0.1000000000000000472, 0.003490658503988666988 ) ;
#9658=DIRECTION ( 'NONE',  ( 0.000000000000000000, 0.000000000000000000, 1.000000000000000000 ) ) ;
#9659=CIRCLE ( 'NONE', #103670, 0.09999999999999982514 ) ;
#9660=EDGE_LOOP ( 'NONE', ( #103057, #29266 ) ) ;
#9661=ORIENTED_EDGE ( 'NONE', *, *, #80016, .F. ) ;
#9662=VERTEX_POINT ( 'NONE', #22771 ) ;
#9663=ORIENTED_EDGE ( 'NONE', *, *, #16748, .F. ) ;
#9664=CARTESIAN_POINT ( 'NONE',  ( 3.149999999999942624, 12.50000000000000000, 6.841600689897072485 ) ) ;
#9665=DIRECTION ( 'NONE',  ( -0.000000000000000000, -1.000000000000000000, -0.000000000000000000 ) ) ;
#9666=FACE_BOUND ( 'NONE', #70858, .T. ) ;
#9667=AXIS2_PLACEMENT_3D ( 'NONE', #34620, #17518, #114433 ) ;
#9668=DIRECTION ( 'NONE',  ( 0.000000000000000000, 0.000000000000000000, -1.000000000000000000 ) ) ;
#9669=CIRCLE ( 'NONE', #49403, 0.06509327318403745899 ) ;
#9670=AXIS2_PLACEMENT_3D ( 'NONE', #71500, #111412, #81963 ) ;
#9671=ORIENTED_EDGE ( 'NONE', *, *, #98562, .F. ) ;
#9672=DIRECTION ( 'NONE',  ( 0.000000000000000000, -0.9999939076577903929, 0.003490651415223739937 ) ) ;
#9673=CARTESIAN_POINT ( 'NONE',  ( 1.249999999999952038, 2.500000000000000000, 2.857883832488649301 ) ) ;
#9674=CARTESIAN_POINT ( 'NONE',  ( 9.149999999999916866, 2.500000000000000000, 7.188010851410848723 ) ) ;
#9675=DIRECTION ( 'NONE',  ( -0.000000000000000000, -1.000000000000000000, -0.000000000000000000 ) ) ;
#9676=ORIENTED_EDGE ( 'NONE', *, *, #112270, .F. ) ;
#9677=DIRECTION ( 'NONE',  ( 0.000000000000000000, 0.000000000000000000, 1.000000000000000000 ) ) ;
#9678=ADVANCED_FACE ( 'NONE', ( #43065 ), #50933, .T. ) ;
#9679=VERTEX_POINT ( 'NONE', #82325 ) ;
#9680=EDGE_CURVE ( 'NONE', #41032, #60331, #73140, .T. ) ;
#9681=ORIENTED_EDGE ( 'NONE', *, *, #63486, .T. ) ;
#9682=EDGE_CURVE ( 'NONE', #76788, #1255, #52909, .T. ) ;
#9683=DIRECTION ( 'NONE',  ( 0.000000000000000000, 0.000000000000000000, 1.000000000000000000 ) ) ;
#9684=DIRECTION ( 'NONE',  ( -0.000000000000000000, 1.000000000000000000, -0.000000000000000000 ) ) ;
#9685=EDGE_CURVE ( 'NONE', #3071, #74230, #12900, .T. ) ;
#9686=ORIENTED_EDGE ( 'NONE', *, *, #33016, .T. ) ;
#9687=ADVANCED_FACE ( 'NONE', ( #52855 ), #121956, .T. ) ;
#9688=LINE ( 'NONE', #56824, #101190 ) ;
#9689=CARTESIAN_POINT ( 'NONE',  ( -11.05000000000000249, 2.500000000000000000, -6.048780366869523029 ) ) ;
#9690=ORIENTED_EDGE ( 'NONE', *, *, #125934, .F. ) ;
#9691=CARTESIAN_POINT ( 'NONE',  ( 3.149999999999946176, 12.50000000000000000, -1.818653347947325916 ) ) ;
#9692=EDGE_CURVE ( 'NONE', #1314, #102047, #50849, .T. ) ;
#9693=ORIENTED_EDGE ( 'NONE', *, *, #122072, .T. ) ;
#9694=DIRECTION ( 'NONE',  ( 0.000000000000000000, 1.000000000000000000, 0.000000000000000000 ) ) ;
#9695=ORIENTED_EDGE ( 'NONE', *, *, #85223, .T. ) ;
#9696=DIRECTION ( 'NONE',  ( 0.000000000000000000, 1.000000000000000000, 0.000000000000000000 ) ) ;
#9697=FACE_BOUND ( 'NONE', #95872, .T. ) ;
#9698=ADVANCED_FACE ( 'NONE', ( #2443 ), #93424, .T. ) ;
#9699=EDGE_CURVE ( 'NONE', #27344, #65690, #100646, .T. ) ;
#9700=VECTOR ( 'NONE', #127697, 1000.000000000000000 ) ;
#9701=EDGE_LOOP ( 'NONE', ( #74981, #73284 ) ) ;
#9702=AXIS2_PLACEMENT_3D ( 'NONE', #74637, #35373, #95575 ) ;
#9703=DIRECTION ( 'NONE',  ( -0.000000000000000000, 1.000000000000000000, -0.000000000000000000 ) ) ;
#9704=ORIENTED_EDGE ( 'NONE', *, *, #89209, .F. ) ;
#9705=CARTESIAN_POINT ( 'NONE',  ( 5.649999999999936406, 2.500000000000000000, -6.148780366869526226 ) ) ;
#9706=CARTESIAN_POINT ( 'NONE',  ( -8.750000000000007105, 12.50000000000000000, 7.122917578226811486 ) ) ;
#9707=CARTESIAN_POINT ( 'NONE',  ( -11.24999999999996447, 12.50000000000000000, -6.560283801567336148 ) ) ;
#9708=LINE ( 'NONE', #30004, #36191 ) ;
#9709=DIRECTION ( 'NONE',  ( 0.000000000000000000, 0.000000000000000000, -1.000000000000000000 ) ) ;
#9710=EDGE_LOOP ( 'NONE', ( #17713, #116716 ) ) ;
#9711=CONICAL_SURFACE ( 'NONE', #22249, 0.09999999999999999167, 0.003490658503988666988 ) ;
#9712=AXIS2_PLACEMENT_3D ( 'NONE', #3696, #92736, #52799 ) ;
#9713=ORIENTED_EDGE ( 'NONE', *, *, #107997, .F. ) ;
#9714=ORIENTED_EDGE ( 'NONE', *, *, #57353, .F. ) ;
#9715=CARTESIAN_POINT ( 'NONE',  ( -11.25000000000000000, 2.500000000000000000, -2.857883832488649745 ) ) ;
#9716=DIRECTION ( 'NONE',  ( 0.000000000000000000, 0.000000000000000000, 1.000000000000000000 ) ) ;
#9717=DIRECTION ( 'NONE',  ( 0.000000000000000000, 1.000000000000000000, 0.000000000000000000 ) ) ;
#9719=ORIENTED_EDGE ( 'NONE', *, *, #58265, .T. ) ;
#9720=ORIENTED_EDGE ( 'NONE', *, *, #110180, .T. ) ;
#9721=DIRECTION ( 'NONE',  ( 0.000000000000000000, 1.000000000000000000, 0.000000000000000000 ) ) ;
#9722=CONICAL_SURFACE ( 'NONE', #11853, 0.1000000000000002554, 0.003490658503988666988 ) ;
#9723=AXIS2_PLACEMENT_3D ( 'NONE', #87861, #8650, #59074 ) ;
#9724=DIRECTION ( 'NONE',  ( 0.000000000000000000, -0.000000000000000000, 1.000000000000000000 ) ) ;
#9725=AXIS2_PLACEMENT_3D ( 'NONE', #112598, #123672, #124350 ) ;
#9727=DIRECTION ( 'NONE',  ( 0.000000000000000000, -0.000000000000000000, 1.000000000000000000 ) ) ;
#9728=LINE ( 'NONE', #69939, #33605 ) ;
#9729=CARTESIAN_POINT ( 'NONE',  ( 8.549999999999918998, 2.500000000000000000, 6.741600689897071952 ) ) ;
#9731=DIRECTION ( 'NONE',  ( 0.000000000000000000, -0.9999939076577903929, 0.003490651415223739937 ) ) ;
#9732=DIRECTION ( 'NONE',  ( 0.000000000000000000, -0.000000000000000000, 1.000000000000000000 ) ) ;
#9733=EDGE_LOOP ( 'NONE', ( #12367, #52725, #112623, #38120 ) ) ;
#9734=EDGE_LOOP ( 'NONE', ( #128776, #111263 ) ) ;
#9735=DIRECTION ( 'NONE',  ( 0.000000000000000000, 1.000000000000000000, 0.000000000000000000 ) ) ;
#9736=DIRECTION ( 'NONE',  ( 0.000000000000000000, 1.000000000000000000, 0.000000000000000000 ) ) ;
#9737=VERTEX_POINT ( 'NONE', #111778 ) ;
#9740=CARTESIAN_POINT ( 'NONE',  ( -0.2000000000000412836, 2.500000000000000000, 4.676537180435972552 ) ) ;
#9741=CONICAL_SURFACE ( 'NONE', #47305, 0.1000000000000002554, 0.003490658503988666988 ) ;
#9742=LINE ( 'NONE', #49688, #56177 ) ;
#9743=CONICAL_SURFACE ( 'NONE', #7663, 0.1000000000000002554, 0.003490658503988666988 ) ;
#9744=DIRECTION ( 'NONE',  ( 0.000000000000000000, 0.000000000000000000, -1.000000000000000000 ) ) ;
#9745=ADVANCED_FACE ( 'NONE', ( #62041 ), #27858, .T. ) ;
#9746=DIRECTION ( 'NONE',  ( -0.000000000000000000, -1.000000000000000000, -0.000000000000000000 ) ) ;
#9747=AXIS2_PLACEMENT_3D ( 'NONE', #117455, #129277, #57943 ) ;
#9748=DIRECTION ( 'NONE',  ( 0.000000000000000000, 0.000000000000000000, -1.000000000000000000 ) ) ;
#9749=CARTESIAN_POINT ( 'NONE',  ( -7.500000000000011546, 12.50000000000000000, 3.702399969078682407 ) ) ;
#9750=AXIS2_PLACEMENT_3D ( 'NONE', #15773, #66167, #5944 ) ;
#9751=CIRCLE ( 'NONE', #68327, 0.1000000000000002554 ) ;
#9752=DIRECTION ( 'NONE',  ( 0.000000000000000000, 0.000000000000000000, 1.000000000000000000 ) ) ;
#9753=ORIENTED_EDGE ( 'NONE', *, *, #9103, .T. ) ;
#9754=AXIS2_PLACEMENT_3D ( 'NONE', #111895, #124294, #112548 ) ;
#9755=ORIENTED_EDGE ( 'NONE', *, *, #117610, .F. ) ;
#9756=VERTEX_POINT ( 'NONE', #65233 ) ;
#9757=ORIENTED_EDGE ( 'NONE', *, *, #126160, .T. ) ;
#9758=FACE_OUTER_BOUND ( 'NONE', #103387, .T. ) ;
#9759=DIRECTION ( 'NONE',  ( -0.000000000000000000, 1.000000000000000000, -0.000000000000000000 ) ) ;
#9760=CIRCLE ( 'NONE', #66183, 0.1000000000000002554 ) ;
#9761=ORIENTED_EDGE ( 'NONE', *, *, #14671, .F. ) ;
#9762=CARTESIAN_POINT ( 'NONE',  ( 9.799999999999913669, 2.500000000000000000, -3.983716857408426293 ) ) ;
#9763=DIRECTION ( 'NONE',  ( 0.000000000000000000, 0.000000000000000000, 1.000000000000000000 ) ) ;
#9764=AXIS2_PLACEMENT_3D ( 'NONE', #44986, #84892, #124829 ) ;
#9765=AXIS2_PLACEMENT_3D ( 'NONE', #125731, #84540, #124472 ) ;
#9767=DIRECTION ( 'NONE',  ( 0.000000000000000000, 0.000000000000000000, 1.000000000000000000 ) ) ;
#9768=ORIENTED_EDGE ( 'NONE', *, *, #83699, .T. ) ;
#9769=DIRECTION ( 'NONE',  ( 0.000000000000000000, -0.9999939076577903929, 0.003490651415223739937 ) ) ;
#9770=LINE ( 'NONE', #129576, #106379 ) ;
#9771=ORIENTED_EDGE ( 'NONE', *, *, #116023, .T. ) ;
#9772=ORIENTED_EDGE ( 'NONE', *, *, #110161, .T. ) ;
#9773=ORIENTED_EDGE ( 'NONE', *, *, #30941, .F. ) ;
#9774=ORIENTED_EDGE ( 'NONE', *, *, #66681, .F. ) ;
#9775=FACE_OUTER_BOUND ( 'NONE', #68908, .T. ) ;
#9776=FACE_OUTER_BOUND ( 'NONE', #1579, .T. ) ;
#9777=DIRECTION ( 'NONE',  ( 0.000000000000000000, -0.000000000000000000, 1.000000000000000000 ) ) ;
#9778=EDGE_CURVE ( 'NONE', #125732, #27245, #113540, .T. ) ;
#9779=ORIENTED_EDGE ( 'NONE', *, *, #124799, .T. ) ;
#9780=DIRECTION ( 'NONE',  ( 0.000000000000000000, 0.000000000000000000, 1.000000000000000000 ) ) ;
#9781=CARTESIAN_POINT ( 'NONE',  ( 7.099999999999925926, 2.500000000000000000, 0.6928203230275494784 ) ) ;
#9782=EDGE_CURVE ( 'NONE', #98804, #114933, #84291, .T. ) ;
#9783=FACE_OUTER_BOUND ( 'NONE', #5889, .T. ) ;
#9784=DIRECTION ( 'NONE',  ( 0.000000000000000000, 0.000000000000000000, 1.000000000000000000 ) ) ;
#9785=EDGE_CURVE ( 'NONE', #102868, #117684, #38340, .T. ) ;
#9786=EDGE_LOOP ( 'NONE', ( #91625, #23686, #60724, #41252 ) ) ;
#9787=AXIS2_PLACEMENT_3D ( 'NONE', #100799, #19687, #92273 ) ;
#9788=PLANE ( 'NONE',  #79264 ) ;
#9789=VECTOR ( 'NONE', #1872, 1000.000000000000000 ) ;
#9790=ORIENTED_EDGE ( 'NONE', *, *, #94333, .T. ) ;
#9791=ADVANCED_FACE ( 'NONE', ( #46246 ), #5025, .T. ) ;
#9792=EDGE_CURVE ( 'NONE', #115818, #126669, #15321, .T. ) ;
#9793=VERTEX_POINT ( 'NONE', #103889 ) ;
#9794=CARTESIAN_POINT ( 'NONE',  ( 0.8499999999999553468, 2.500000000000000000, -2.857883832488653741 ) ) ;
#9795=ADVANCED_FACE ( 'NONE', ( #96620 ), #82155, .T. ) ;
#9796=LINE ( 'NONE', #98167, #100431 ) ;
#9797=EDGE_CURVE ( 'NONE', #18483, #77736, #24686, .T. ) ;
#9798=FACE_BOUND ( 'NONE', #82594, .T. ) ;
#9800=DIRECTION ( 'NONE',  ( -0.000000000000000000, 1.000000000000000000, -0.000000000000000000 ) ) ;
#9801=AXIS2_PLACEMENT_3D ( 'NONE', #109930, #79810, #119727 ) ;
#9802=AXIS2_PLACEMENT_3D ( 'NONE', #11265, #51218, #803 ) ;
#9803=CARTESIAN_POINT ( 'NONE',  ( 14.14999999999989555, 2.500000000000000000, 2.065063509461097624 ) ) ;
#9804=EDGE_LOOP ( 'NONE', ( #38983, #56572 ) ) ;
#9805=DIRECTION ( 'NONE',  ( -0.000000000000000000, 1.000000000000000000, -0.000000000000000000 ) ) ;
#9806=DIRECTION ( 'NONE',  ( 0.000000000000000000, 0.000000000000000000, 1.000000000000000000 ) ) ;
#9807=VECTOR ( 'NONE', #63634, 1000.000000000000000 ) ;
#9808=ADVANCED_FACE ( 'NONE', ( #54773 ), #75970, .T. ) ;
#9809=DIRECTION ( 'NONE',  ( 0.000000000000000000, 0.000000000000000000, 1.000000000000000000 ) ) ;
#9810=CARTESIAN_POINT ( 'NONE',  ( 1.449999999999951772, 2.500000000000000000, -6.148780366869526226 ) ) ;
#9811=ORIENTED_EDGE ( 'NONE', *, *, #65699, .F. ) ;
#9812=CIRCLE ( 'NONE', #22350, 0.1000000000000002554 ) ;
#9813=DIRECTION ( 'NONE',  ( 0.000000000000000000, 0.000000000000000000, -1.000000000000000000 ) ) ;
#9814=CIRCLE ( 'NONE', #99711, 0.1000000000000000056 ) ;
#9815=DIRECTION ( 'NONE',  ( 0.000000000000000000, 0.000000000000000000, 1.000000000000000000 ) ) ;
#9816=EDGE_LOOP ( 'NONE', ( #35705, #53150, #87910, #56757 ) ) ;
#9817=ORIENTED_EDGE ( 'NONE', *, *, #122609, .F. ) ;
#9818=LINE ( 'NONE', #81767, #60733 ) ;
#9819=CARTESIAN_POINT ( 'NONE',  ( 13.09999999999989839, 12.50000000000000000, -0.3464101615137783474 ) ) ;
#9820=FACE_BOUND ( 'NONE', #71787, .T. ) ;
#9821=LINE ( 'NONE', #110594, #116257 ) ;
#9822=DIRECTION ( 'NONE',  ( 1.000000000000000000, 0.000000000000000000, 0.000000000000000000 ) ) ;
#9823=ORIENTED_EDGE ( 'NONE', *, *, #66936, .F. ) ;
#9824=DIRECTION ( 'NONE',  ( -0.000000000000000000, -1.000000000000000000, -0.000000000000000000 ) ) ;
#9825=EDGE_CURVE ( 'NONE', #10582, #112123, #16765, .T. ) ;
#9827=VERTEX_POINT ( 'NONE', #36458 ) ;
#9828=FACE_OUTER_BOUND ( 'NONE', #115970, .T. ) ;
#9829=DIRECTION ( 'NONE',  ( 0.000000000000000000, 1.000000000000000000, 0.000000000000000000 ) ) ;
#9830=AXIS2_PLACEMENT_3D ( 'NONE', #121354, #53287, #70975 ) ;
#9831=EDGE_CURVE ( 'NONE', #85857, #50468, #104524, .T. ) ;
#9832=ADVANCED_FACE ( 'NONE', ( #125454 ), #76368, .T. ) ;
#9833=DIRECTION ( 'NONE',  ( 0.000000000000000000, 0.000000000000000000, 1.000000000000000000 ) ) ;
#9834=CARTESIAN_POINT ( 'NONE',  ( 9.149999999999916866, 2.500000000000000000, -2.757883832488654097 ) ) ;
#9835=EDGE_CURVE ( 'NONE', #107613, #53181, #124169, .T. ) ;
#9836=AXIS2_PLACEMENT_3D ( 'NONE', #101928, #32564, #24011 ) ;
#9837=VERTEX_POINT ( 'NONE', #94702 ) ;
#9838=AXIS2_PLACEMENT_3D ( 'NONE', #50500, #102196, #90413 ) ;
#9839=EDGE_CURVE ( 'NONE', #55841, #26633, #103165, .T. ) ;
#9840=CARTESIAN_POINT ( 'NONE',  ( 2.899999999999946620, 2.500000000000000000, 0.5928203230275495006 ) ) ;
#9841=CARTESIAN_POINT ( 'NONE',  ( -4.350000000000023626, 12.50000000000000000, -1.883746621131363375 ) ) ;
#9842=DIRECTION ( 'NONE',  ( 0.000000000000000000, 1.000000000000000000, 0.000000000000000000 ) ) ;
#9843=CARTESIAN_POINT ( 'NONE',  ( -10.85000000000000142, 2.500000000000000000, -5.702370205355745902 ) ) ;
#9844=ORIENTED_EDGE ( 'NONE', *, *, #63116, .F. ) ;
#9845=EDGE_LOOP ( 'NONE', ( #69300, #82147 ) ) ;
#9846=CIRCLE ( 'NONE', #76657, 0.1000000000000002554 ) ;
#9847=EDGE_CURVE ( 'NONE', #29739, #21836, #56691, .T. ) ;
#9848=DIRECTION ( 'NONE',  ( 0.000000000000000000, 0.000000000000000000, 1.000000000000000000 ) ) ;
#9849=CONICAL_SURFACE ( 'NONE', #43049, 0.09999999999999982514, 0.003490658503988666988 ) ;
#9850=ADVANCED_FACE ( 'NONE', ( #66528 ), #6942, .T. ) ;
#9851=EDGE_LOOP ( 'NONE', ( #80452, #95524 ) ) ;
#9852=FACE_OUTER_BOUND ( 'NONE', #44801, .T. ) ;
#9853=CARTESIAN_POINT ( 'NONE',  ( -7.900000000000014566, 2.500000000000000000, -4.330127018922201643 ) ) ;
#9854=EDGE_CURVE ( 'NONE', #64742, #92706, #36295, .T. ) ;
#9855=CIRCLE ( 'NONE', #106089, 0.09999999999999982514 ) ;
#9856=AXIS2_PLACEMENT_3D ( 'NONE', #17714, #88385, #126400 ) ;
#9857=EDGE_CURVE ( 'NONE', #1183, #61868, #115676, .T. ) ;
#9858=DIRECTION ( 'NONE',  ( 0.000000000000000000, 0.000000000000000000, 1.000000000000000000 ) ) ;
#9859=ORIENTED_EDGE ( 'NONE', *, *, #16821, .F. ) ;
#9860=DIRECTION ( 'NONE',  ( 0.000000000000000000, 0.000000000000000000, 1.000000000000000000 ) ) ;
#9861=CARTESIAN_POINT ( 'NONE',  ( -12.09999999999999432, 2.500000000000000000, 3.637306695894644726 ) ) ;
#9862=CARTESIAN_POINT ( 'NONE',  ( 0.8499999999999545697, 12.50000000000000000, 2.922977105672686982 ) ) ;
#9863=CARTESIAN_POINT ( 'NONE',  ( -6.050000000000020250, 2.500000000000000000, -2.611473670974877592 ) ) ;
#9864=CARTESIAN_POINT ( 'NONE',  ( -9.999999999999971578, 12.50000000000000000, -4.330127018922197202 ) ) ;
#9865=CARTESIAN_POINT ( 'NONE',  ( 3.099999999999945466, 2.500000000000000000, 0.3464101615137735735 ) ) ;
#9866=ADVANCED_FACE ( 'NONE', ( #18072 ), #46742, .T. ) ;
#9867=ORIENTED_EDGE ( 'NONE', *, *, #3436, .F. ) ;
#9868=EDGE_LOOP ( 'NONE', ( #10515, #71762 ) ) ;
#9869=DIRECTION ( 'NONE',  ( 0.000000000000000000, -0.000000000000000000, 1.000000000000000000 ) ) ;
#9870=ORIENTED_EDGE ( 'NONE', *, *, #92905, .F. ) ;
#9872=EDGE_LOOP ( 'NONE', ( #35421, #4507, #38197, #15860 ) ) ;
#9873=ORIENTED_EDGE ( 'NONE', *, *, #3292, .T. ) ;
#9874=VERTEX_POINT ( 'NONE', #78955 ) ;
#9875=VECTOR ( 'NONE', #127392, 1000.000000000000000 ) ;
#9876=DIRECTION ( 'NONE',  ( 0.000000000000000000, 1.000000000000000000, 0.000000000000000000 ) ) ;
#9877=PLANE ( 'NONE',  #77838 ) ;
#9880=DIRECTION ( 'NONE',  ( -0.000000000000000000, 1.000000000000000000, -0.000000000000000000 ) ) ;
#9881=CARTESIAN_POINT ( 'NONE',  ( 4.799999999999937650, 2.500000000000000000, -4.083716857408426826 ) ) ;
#9882=DIRECTION ( 'NONE',  ( 0.000000000000000000, 0.000000000000000000, 1.000000000000000000 ) ) ;
#9883=CARTESIAN_POINT ( 'NONE',  ( 9.999999999999948486, 12.50000000000000000, -4.330127018922201643 ) ) ;
#9884=DIRECTION ( 'NONE',  ( -0.000000000000000000, 1.000000000000000000, -0.000000000000000000 ) ) ;
#9885=CARTESIAN_POINT ( 'NONE',  ( 8.949999999999915801, 2.500000000000000000, 6.841600689897072485 ) ) ;
#9886=ORIENTED_EDGE ( 'NONE', *, *, #77039, .T. ) ;
#9887=CIRCLE ( 'NONE', #76786, 0.1000000000000000472 ) ;
#9888=VERTEX_POINT ( 'NONE', #48849 ) ;
#9889=CONICAL_SURFACE ( 'NONE', #14066, 0.1000000000000002554, 0.003490658503988666988 ) ;
#9890=FACE_OUTER_BOUND ( 'NONE', #88075, .T. ) ;
#9892=ORIENTED_EDGE ( 'NONE', *, *, #749, .F. ) ;
#9894=AXIS2_PLACEMENT_3D ( 'NONE', #9629, #89480, #129437 ) ;
#9895=CIRCLE ( 'NONE', #112310, 0.1000000000000000056 ) ;
#9896=DIRECTION ( 'NONE',  ( 0.000000000000000000, 1.000000000000000000, 0.000000000000000000 ) ) ;
#9897=CIRCLE ( 'NONE', #99785, 0.06509327318403745899 ) ;
#9898=EDGE_CURVE ( 'NONE', #32791, #31641, #69720, .T. ) ;
#9899=CARTESIAN_POINT ( 'NONE',  ( 12.94999999999990337, 2.500000000000000000, 2.065063509461097624 ) ) ;
#9900=CARTESIAN_POINT ( 'NONE',  ( -13.34999999999999076, 12.50000000000000000, -2.230156782645137170 ) ) ;
#9901=LINE ( 'NONE', #717, #101114 ) ;
#9902=ORIENTED_EDGE ( 'NONE', *, *, #115815, .F. ) ;
#9903=AXIS2_PLACEMENT_3D ( 'NONE', #111887, #82444, #9815 ) ;
#9904=EDGE_LOOP ( 'NONE', ( #34686, #50514, #114934, #75756 ) ) ;
#9905=CARTESIAN_POINT ( 'NONE',  ( 1.049999999999953637, 12.50000000000000000, 2.511473670974873507 ) ) ;
#9906=CONICAL_SURFACE ( 'NONE', #81009, 0.1000000000000002554, 0.003490658503988666988 ) ;
#9908=DIRECTION ( 'NONE',  ( -4.274815082592931898E-19, -0.9999939076577903929, -0.003490651415223739937 ) ) ;
#9909=ORIENTED_EDGE ( 'NONE', *, *, #9680, .T. ) ;
#9910=EDGE_CURVE ( 'NONE', #22838, #25337, #19543, .T. ) ;
#9911=ORIENTED_EDGE ( 'NONE', *, *, #3505, .F. ) ;
#9912=CARTESIAN_POINT ( 'NONE',  ( -3.750000000000029310, 2.500000000000000000, -7.188010851410854052 ) ) ;
#9913=FACE_OUTER_BOUND ( 'NONE', #67963, .T. ) ;
#9914=DIRECTION ( 'NONE',  ( 0.000000000000000000, 0.000000000000000000, -1.000000000000000000 ) ) ;
#9915=DIRECTION ( 'NONE',  ( -0.000000000000000000, -1.000000000000000000, -0.000000000000000000 ) ) ;
#9917=DIRECTION ( 'NONE',  ( -0.000000000000000000, 1.000000000000000000, -0.000000000000000000 ) ) ;
#9918=ORIENTED_EDGE ( 'NONE', *, *, #107806, .F. ) ;
#9919=DIRECTION ( 'NONE',  ( -0.000000000000000000, 1.000000000000000000, -0.000000000000000000 ) ) ;
#9920=PLANE ( 'NONE',  #82889 ) ;
#9921=CARTESIAN_POINT ( 'NONE',  ( 3.299999999999942979, 12.50000000000000000, 4.395220292106234439 ) ) ;
#9922=CARTESIAN_POINT ( 'NONE',  ( -12.89999999999999147, 2.500000000000000000, 1.843143693225357538E-15 ) ) ;
#9923=AXIS2_PLACEMENT_3D ( 'NONE', #44466, #115784, #94213 ) ;
#9924=AXIS2_PLACEMENT_3D ( 'NONE', #117884, #17749, #97609 ) ;
#9925=DIRECTION ( 'NONE',  ( 0.000000000000000000, 0.000000000000000000, 1.000000000000000000 ) ) ;
#9926=VERTEX_POINT ( 'NONE', #98550 ) ;
#9927=CONICAL_SURFACE ( 'NONE', #20398, 0.1000000000000000056, 0.003490658503988666988 ) ;
#9928=ORIENTED_EDGE ( 'NONE', *, *, #124499, .T. ) ;
#9929=DIRECTION ( 'NONE',  ( -0.000000000000000000, -1.000000000000000000, -0.000000000000000000 ) ) ;
#9930=AXIS2_PLACEMENT_3D ( 'NONE', #2934, #2259, #43512 ) ;
#9931=EDGE_LOOP ( 'NONE', ( #102016, #31362 ) ) ;
#9932=AXIS2_PLACEMENT_3D ( 'NONE', #122701, #61861, #103052 ) ;
#9933=CARTESIAN_POINT ( 'NONE',  ( 17.17279024593006298, -1.352253750625425743, 5.266180533622979887 ) ) ;
#9934=CARTESIAN_POINT ( 'NONE',  ( 0.3999999999999619971, 2.500000000000000000, -1.084202172485504434E-16 ) ) ;
#9935=CIRCLE ( 'NONE', #112343, 0.1000000000000002554 ) ;
#9936=EDGE_CURVE ( 'NONE', #122938, #68683, #69761, .T. ) ;
#9937=VERTEX_POINT ( 'NONE', #97285 ) ;
#9938=DIRECTION ( 'NONE',  ( 0.000000000000000000, -0.9999939076577903929, 0.003490651415223739937 ) ) ;
#9939=DIRECTION ( 'NONE',  ( -0.000000000000000000, 1.000000000000000000, -0.000000000000000000 ) ) ;
#9940=CIRCLE ( 'NONE', #16175, 0.06509327318403743123 ) ;
#9941=CARTESIAN_POINT ( 'NONE',  ( -6.850000000000013856, 12.50000000000000000, 2.576566944158910744 ) ) ;
#9942=DIRECTION ( 'NONE',  ( 0.000000000000000000, 0.000000000000000000, 1.000000000000000000 ) ) ;
#9944=AXIS2_PLACEMENT_3D ( 'NONE', #25661, #76061, #74135 ) ;
#9945=CIRCLE ( 'NONE', #122817, 0.1000000000000002554 ) ;
#9946=LINE ( 'NONE', #40056, #20579 ) ;
#9947=EDGE_LOOP ( 'NONE', ( #73728, #26402 ) ) ;
#9948=EDGE_CURVE ( 'NONE', #126006, #36337, #69149, .T. ) ;
#9949=ADVANCED_FACE ( 'NONE', ( #87453 ), #71221, .T. ) ;
#9950=EDGE_CURVE ( 'NONE', #120872, #43692, #77632, .T. ) ;
#9951=CARTESIAN_POINT ( 'NONE',  ( 21.15177371151417773, 2.593223176056361545, -4.151029080743465549 ) ) ;
#9952=ADVANCED_FACE ( 'NONE', ( #59977 ), #64952, .T. ) ;
#9953=EDGE_CURVE ( 'NONE', #6356, #47855, #35718, .T. ) ;
#9954=DIRECTION ( 'NONE',  ( 0.000000000000000000, 1.000000000000000000, 0.000000000000000000 ) ) ;
#9955=CARTESIAN_POINT ( 'NONE',  ( 2.099999999999949463, 12.50000000000000000, 0.6928203230275494784 ) ) ;
#9956=ORIENTED_EDGE ( 'NONE', *, *, #118438, .T. ) ;
#9957=CARTESIAN_POINT ( 'NONE',  ( -4.600000000000024514, 12.50000000000000000, 3.572213422710607489 ) ) ;
#9958=ORIENTED_EDGE ( 'NONE', *, *, #110883, .F. ) ;
#9959=DIRECTION ( 'NONE',  ( -0.000000000000000000, 1.000000000000000000, -0.000000000000000000 ) ) ;
#9960=DIRECTION ( 'NONE',  ( 0.000000000000000000, 1.000000000000000000, 0.000000000000000000 ) ) ;
#9961=VECTOR ( 'NONE', #16252, 1000.000000000000000 ) ;
#9962=EDGE_CURVE ( 'NONE', #22161, #98907, #81686, .T. ) ;
#9963=CARTESIAN_POINT ( 'NONE',  ( -4.076600168545496672E-14, 12.50000000000000000, -5.022947341949754119 ) ) ;
#9964=ORIENTED_EDGE ( 'NONE', *, *, #98410, .T. ) ;
#9965=EDGE_CURVE ( 'NONE', #1501, #114265, #108864, .T. ) ;
#9966=CARTESIAN_POINT ( 'NONE',  ( 3.349999999999943689, 2.500000000000000000, 1.472243186433545459 ) ) ;
#9967=EDGE_CURVE ( 'NONE', #33641, #105724, #52433, .T. ) ;
#9968=CARTESIAN_POINT ( 'NONE',  ( 0.8499999999999553468, 2.500000000000000000, 1.572243186433545548 ) ) ;
#9969=ORIENTED_EDGE ( 'NONE', *, *, #122375, .F. ) ;
#9970=DIRECTION ( 'NONE',  ( -0.000000000000000000, 1.000000000000000000, -0.000000000000000000 ) ) ;
#9971=ORIENTED_EDGE ( 'NONE', *, *, #103662, .T. ) ;
#9973=AXIS2_PLACEMENT_3D ( 'NONE', #10044, #117382, #49344 ) ;
#9975=ORIENTED_EDGE ( 'NONE', *, *, #115747, .T. ) ;
#9976=FACE_OUTER_BOUND ( 'NONE', #107554, .T. ) ;
#9977=LINE ( 'NONE', #19801, #91918 ) ;
#9978=EDGE_LOOP ( 'NONE', ( #108802, #47738 ) ) ;
#9979=ORIENTED_EDGE ( 'NONE', *, *, #2687, .T. ) ;
#9980=CARTESIAN_POINT ( 'NONE',  ( -5.400000000000019895, 2.500000000000000000, 0.09999999999999772959 ) ) ;
#9981=DIRECTION ( 'NONE',  ( 0.000000000000000000, 1.000000000000000000, 0.000000000000000000 ) ) ;
#9982=EDGE_LOOP ( 'NONE', ( #37754, #39301, #85937, #82280 ) ) ;
#9983=CIRCLE ( 'NONE', #79051, 0.06509327318403745899 ) ;
#9984=CARTESIAN_POINT ( 'NONE',  ( 5.649999999999936406, 12.50000000000000000, -6.148780366869526226 ) ) ;
#9986=CONICAL_SURFACE ( 'NONE', #58120, 0.1000000000000000472, 0.003490658503988666988 ) ;
#9987=CONICAL_SURFACE ( 'NONE', #10274, 0.1000000000000000472, 0.003490658503988666988 ) ;
#9990=LINE ( 'NONE', #19136, #86451 ) ;
#9991=CARTESIAN_POINT ( 'NONE',  ( 5.399999999999935518, 2.500000000000000000, -4.430127018922202176 ) ) ;
#9992=CARTESIAN_POINT ( 'NONE',  ( -8.749999999999975131, 12.50000000000000000, -2.165063509461101710 ) ) ;
#9993=AXIS2_PLACEMENT_3D ( 'NONE', #27528, #67437, #30792 ) ;
#9994=EDGE_LOOP ( 'NONE', ( #124785, #27878 ) ) ;
#9995=ORIENTED_EDGE ( 'NONE', *, *, #82182, .F. ) ;
#9996=VERTEX_POINT ( 'NONE', #58661 ) ;
#9997=EDGE_LOOP ( 'NONE', ( #24205, #115791 ) ) ;
#9998=DIRECTION ( 'NONE',  ( 0.000000000000000000, 0.000000000000000000, 1.000000000000000000 ) ) ;
#9999=DIRECTION ( 'NONE',  ( 0.000000000000000000, 0.000000000000000000, 1.000000000000000000 ) ) ;
#10000=AXIS2_PLACEMENT_3D ( 'NONE', #48079, #38926, #117417 ) ;
#10001=CARTESIAN_POINT ( 'NONE',  ( -5.600000000000023626, 2.500000000000000000, -3.983716857408426293 ) ) ;
#10002=ORIENTED_EDGE ( 'NONE', *, *, #45262, .T. ) ;
#10003=FACE_BOUND ( 'NONE', #56246, .T. ) ;
#10004=VERTEX_POINT ( 'NONE', #28556 ) ;
#10005=ADVANCED_FACE ( 'NONE', ( #68460 ), #88760, .T. ) ;
#10006=DIRECTION ( 'NONE',  ( 0.000000000000000000, 0.000000000000000000, 1.000000000000000000 ) ) ;
#10007=CARTESIAN_POINT ( 'NONE',  ( -1.250000000000001110, 2.500000000000000000, -6.595190528383302109 ) ) ;
#10008=ADVANCED_FACE ( 'NONE', ( #109020 ), #110998, .T. ) ;
#10009=CARTESIAN_POINT ( 'NONE',  ( 1.649999999999948841, 12.50000000000000000, 6.495190528383297135 ) ) ;
#10010=CIRCLE ( 'NONE', #30957, 0.06509327318403745899 ) ;
#10011=FACE_OUTER_BOUND ( 'NONE', #10972, .T. ) ;
#10012=ADVANCED_FACE ( 'NONE', ( #27248 ), #115104, .T. ) ;
#10013=CARTESIAN_POINT ( 'NONE',  ( -5.850000000000018296, 2.500000000000000000, 7.188010851410848723 ) ) ;
#10015=CARTESIAN_POINT ( 'NONE',  ( -7.700000000000016165, 2.500000000000000000, 0.3464101615137735735 ) ) ;
#10016=DIRECTION ( 'NONE',  ( 0.000000000000000000, 1.000000000000000000, 0.000000000000000000 ) ) ;
#10017=DIRECTION ( 'NONE',  ( 0.000000000000000000, 1.000000000000000000, 0.000000000000000000 ) ) ;
#10018=VECTOR ( 'NONE', #49341, 1000.000000000000000 ) ;
#10019=CARTESIAN_POINT ( 'NONE',  ( -5.850000000000022737, 12.50000000000000000, -6.495190528383302464 ) ) ;
#10020=EDGE_CURVE ( 'NONE', #28942, #124332, #125583, .T. ) ;
#10021=ORIENTED_EDGE ( 'NONE', *, *, #98158, .F. ) ;
#10022=CONICAL_SURFACE ( 'NONE', #56065, 0.1000000000000002554, 0.003490658503988666988 ) ;
#10023=ORIENTED_EDGE ( 'NONE', *, *, #65325, .F. ) ;
#10024=EDGE_LOOP ( 'NONE', ( #3052, #91029, #94387, #5564 ) ) ;
#10026=DIRECTION ( 'NONE',  ( 0.000000000000000000, 1.000000000000000000, 0.000000000000000000 ) ) ;
#10027=CARTESIAN_POINT ( 'NONE',  ( 3.549999999999944755, 2.500000000000000000, -6.841600689897077814 ) ) ;
#10028=ORIENTED_EDGE ( 'NONE', *, *, #78258, .T. ) ;
#10029=ORIENTED_EDGE ( 'NONE', *, *, #45778, .T. ) ;
#10030=VECTOR ( 'NONE', #26438, 1000.000000000000000 ) ;
#10031=ORIENTED_EDGE ( 'NONE', *, *, #72682, .T. ) ;
#10033=AXIS2_PLACEMENT_3D ( 'NONE', #29182, #29812, #117504 ) ;
#10034=AXIS2_PLACEMENT_3D ( 'NONE', #54850, #93506, #34610 ) ;
#10035=DIRECTION ( 'NONE',  ( -0.000000000000000000, 1.000000000000000000, -0.000000000000000000 ) ) ;
#10036=CARTESIAN_POINT ( 'NONE',  ( -8.950000000000008171, 12.50000000000000000, 1.818653347947321475 ) ) ;
#10037=DIRECTION ( 'NONE',  ( 0.000000000000000000, 0.000000000000000000, 1.000000000000000000 ) ) ;
#10038=CARTESIAN_POINT ( 'NONE',  ( 7.299999999999926104, 2.500000000000000000, 4.676537180435972552 ) ) ;
#10040=DIRECTION ( 'NONE',  ( -4.274815082592931898E-19, -0.9999939076577903929, -0.003490651415223739937 ) ) ;
#10041=AXIS2_PLACEMENT_3D ( 'NONE', #17421, #57370, #107757 ) ;
#10042=ADVANCED_FACE ( 'NONE', ( #93272 ), #12711, .T. ) ;
#10043=EDGE_LOOP ( 'NONE', ( #80725, #110389, #109277, #8163 ) ) ;
#10044=CARTESIAN_POINT ( 'NONE',  ( 4.799999999999939426, 2.500000000000000000, -4.676537180435977881 ) ) ;
#10045=VERTEX_POINT ( 'NONE', #112278 ) ;
#10046=CIRCLE ( 'NONE', #85254, 0.06509327318403745899 ) ;
#10047=AXIS2_PLACEMENT_3D ( 'NONE', #99861, #98534, #69742 ) ;
#10048=ORIENTED_EDGE ( 'NONE', *, *, #29335, .F. ) ;
#10049=EDGE_LOOP ( 'NONE', ( #3958, #78134 ) ) ;
#10050=LINE ( 'NONE', #110812, #121623 ) ;
#10051=( BOUNDED_SURFACE ( )  B_SPLINE_SURFACE ( 3, 2, ( 
 ( #128578, #59839, #50625 ),
 ( #120020, #129220, #88621 ),
 ( #9420, #31017, #118073 ),
 ( #108254, #110200, #90547 ) ),
 .UNSPECIFIED., .F., .F., .F. ) 
 B_SPLINE_SURFACE_WITH_KNOTS ( ( 4, 4 ),
 ( 3, 3 ),
 ( 0.02228103309872378826, 0.02393870366795248020 ),
 ( 0.000000000000000000, 1.000000000000000000 ),
 .UNSPECIFIED. ) 
 GEOMETRIC_REPRESENTATION_ITEM ( )  RATIONAL_B_SPLINE_SURFACE ( (
 ( 1.000000000000000000, 0.9066952437723002634, 1.000000000000000000),
 ( 1.000000000000000000, 0.9065452688549063831, 1.000000000000000000),
 ( 1.000000000000000000, 0.9065452844449193304, 1.000000000000000000),
 ( 1.000000000000000000, 0.9066952434955795059, 1.000000000000000000) ) ) 
 REPRESENTATION_ITEM ( '' )  SURFACE ( )  );
#10052=ORIENTED_EDGE ( 'NONE', *, *, #14633, .F. ) ;
#10053=ORIENTED_EDGE ( 'NONE', *, *, #44334, .T. ) ;
#10054=CARTESIAN_POINT ( 'NONE',  ( 9.149999999999916866, 12.50000000000000000, -2.857883832488653741 ) ) ;
#10055=FACE_OUTER_BOUND ( 'NONE', #79138, .T. ) ;
#10056=CARTESIAN_POINT ( 'NONE',  ( -10.00000000000000533, 2.500000000000000000, -5.022947341949749678 ) ) ;
#10057=ADVANCED_FACE ( 'NONE', ( #30508 ), #14753, .T. ) ;
#10058=DIRECTION ( 'NONE',  ( -0.000000000000000000, 1.000000000000000000, -0.000000000000000000 ) ) ;
#10060=EDGE_LOOP ( 'NONE', ( #72756, #66283, #22042, #43302 ) ) ;
#10061=LINE ( 'NONE', #18588, #99330 ) ;
#10062=ORIENTED_EDGE ( 'NONE', *, *, #1024, .T. ) ;
#10063=PLANE ( 'NONE',  #81785 ) ;
#10064=EDGE_LOOP ( 'NONE', ( #129156, #35746 ) ) ;
#10066=PLANE ( 'NONE',  #90904 ) ;
#10067=CIRCLE ( 'NONE', #35211, 0.09999999999999982514 ) ;
#10068=ORIENTED_EDGE ( 'NONE', *, *, #95970, .T. ) ;
#10070=AXIS2_PLACEMENT_3D ( 'NONE', #32572, #53486, #22104 ) ;
#10071=ADVANCED_FACE ( 'NONE', ( #111621 ), #197, .T. ) ;
#10072=CARTESIAN_POINT ( 'NONE',  ( 3.349999999999941913, 12.50000000000000000, 5.802370205355744659 ) ) ;
#10073=VERTEX_POINT ( 'NONE', #22617 ) ;
#10074=AXIS2_PLACEMENT_3D ( 'NONE', #53094, #21045, #760 ) ;
#10075=LINE ( 'NONE', #8759, #115562 ) ;
#10076=ORIENTED_EDGE ( 'NONE', *, *, #81200, .F. ) ;
#10077=EDGE_LOOP ( 'NONE', ( #84665, #82895 ) ) ;
#10078=DIRECTION ( 'NONE',  ( 0.000000000000000000, 0.000000000000000000, 1.000000000000000000 ) ) ;
#10079=DIRECTION ( 'NONE',  ( 0.000000000000000000, 1.000000000000000000, 0.000000000000000000 ) ) ;
#10081=LINE ( 'NONE', #50031, #78588 ) ;
#10082=AXIS2_PLACEMENT_3D ( 'NONE', #89494, #68554, #129450 ) ;
#10083=CARTESIAN_POINT ( 'NONE',  ( 13.14999999999989733, 2.500000000000000000, -2.511473670974877948 ) ) ;
#10084=CIRCLE ( 'NONE', #97897, 0.1000000000000002554 ) ;
#10085=ORIENTED_EDGE ( 'NONE', *, *, #82061, .T. ) ;
#10086=CARTESIAN_POINT ( 'NONE',  ( 5.649999999999934630, 2.500000000000000000, -2.411473670974877859 ) ) ;
#10087=ORIENTED_EDGE ( 'NONE', *, *, #26743, .F. ) ;
#10088=DIRECTION ( 'NONE',  ( 0.000000000000000000, -0.9999939076577903929, 0.003490651415223739937 ) ) ;
#10089=CARTESIAN_POINT ( 'NONE',  ( -11.64999999999999680, 2.500000000000000000, 1.372243186433545370 ) ) ;
#10090=AXIS2_PLACEMENT_3D ( 'NONE', #18207, #17561, #126892 ) ;
#10091=EDGE_CURVE ( 'NONE', #127944, #16485, #43543, .T. ) ;
#10092=VECTOR ( 'NONE', #17794, 1000.000000000000000 ) ;
#10094=PLANE ( 'NONE',  #40583 ) ;
#10095=CARTESIAN_POINT ( 'NONE',  ( -6.650000000000015454, 2.500000000000000000, 7.288010851410849256 ) ) ;
#10098=EDGE_LOOP ( 'NONE', ( #101218, #32105 ) ) ;
#10099=ADVANCED_FACE ( 'NONE', ( #42245 ), #62905, .T. ) ;
#10100=CIRCLE ( 'NONE', #18499, 0.1000000000000002554 ) ;
#10101=LINE ( 'NONE', #108924, #56385 ) ;
#10103=DIRECTION ( 'NONE',  ( -0.000000000000000000, 1.000000000000000000, -0.000000000000000000 ) ) ;
#10105=ADVANCED_FACE ( 'NONE', ( #51432 ), #75418, .T. ) ;
#10106=EDGE_CURVE ( 'NONE', #126067, #65404, #87926, .T. ) ;
#10107=ADVANCED_FACE ( 'NONE', ( #120791 ), #23187, .T. ) ;
#10108=EDGE_CURVE ( 'NONE', #106239, #27297, #123534, .T. ) ;
#10109=ORIENTED_EDGE ( 'NONE', *, *, #20277, .T. ) ;
#10110=AXIS2_PLACEMENT_3D ( 'NONE', #121436, #71701, #40978 ) ;
#10111=CARTESIAN_POINT ( 'NONE',  ( 2.099999999999950351, 2.500000000000000000, -4.330127018922201643 ) ) ;
#10112=ORIENTED_EDGE ( 'NONE', *, *, #7997, .T. ) ;
#10113=VERTEX_POINT ( 'NONE', #110952 ) ;
#10114=DIRECTION ( 'NONE',  ( 0.000000000000000000, 0.000000000000000000, -1.000000000000000000 ) ) ;
#10115=EDGE_CURVE ( 'NONE', #68058, #98606, #67073, .T. ) ;
#10116=EDGE_CURVE ( 'NONE', #83265, #8819, #56620, .T. ) ;
#10117=EDGE_LOOP ( 'NONE', ( #50682, #117539 ) ) ;
#10118=CIRCLE ( 'NONE', #1780, 0.06509327318403745899 ) ;
#10119=CARTESIAN_POINT ( 'NONE',  ( 6.699999999999928235, 2.500000000000000000, 0.09999999999999772959 ) ) ;
#10120=LINE ( 'NONE', #40223, #13025 ) ;
#10121=EDGE_CURVE ( 'NONE', #37337, #1478, #54492, .T. ) ;
#10122=ORIENTED_EDGE ( 'NONE', *, *, #112026, .T. ) ;
#10123=EDGE_CURVE ( 'NONE', #527, #70003, #48237, .T. ) ;
#10124=CARTESIAN_POINT ( 'NONE',  ( -7.700000000000010836, 12.50000000000000000, 3.983716857408420964 ) ) ;
#10125=EDGE_CURVE ( 'NONE', #107157, #11464, #52696, .T. ) ;
#10126=FACE_OUTER_BOUND ( 'NONE', #66385, .T. ) ;
#10127=CARTESIAN_POINT ( 'NONE',  ( -5.450000000000023270, 12.50000000000000000, -2.230156782645139391 ) ) ;
#10129=EDGE_CURVE ( 'NONE', #99984, #65002, #98399, .T. ) ;
#10130=ORIENTED_EDGE ( 'NONE', *, *, #71145, .F. ) ;
#10131=CIRCLE ( 'NONE', #31001, 0.1000000000000002554 ) ;
#10132=CONICAL_SURFACE ( 'NONE', #45650, 0.1000000000000002554, 0.003490658503988666988 ) ;
#10133=ORIENTED_EDGE ( 'NONE', *, *, #59203, .F. ) ;
#10134=ORIENTED_EDGE ( 'NONE', *, *, #66099, .T. ) ;
#10135=CARTESIAN_POINT ( 'NONE',  ( 5.399999999999933742, 2.500000000000000000, -0.1000000000000023925 ) ) ;
#10136=CARTESIAN_POINT ( 'NONE',  ( 7.899999999999924860, 2.500000000000000000, 3.637306695894644726 ) ) ;
#10137=CARTESIAN_POINT ( 'NONE',  ( -3.300000000000027800, 12.50000000000000000, -4.265033745738164406 ) ) ;
#10138=FACE_BOUND ( 'NONE', #51115, .T. ) ;
#10139=VERTEX_POINT ( 'NONE', #82163 ) ;
#10140=DIRECTION ( 'NONE',  ( 0.000000000000000000, 0.000000000000000000, 1.000000000000000000 ) ) ;
#10141=CARTESIAN_POINT ( 'NONE',  ( 12.89999999999990266, 2.500000000000000000, 3.737306695894644371 ) ) ;
#10142=ORIENTED_EDGE ( 'NONE', *, *, #117137, .F. ) ;
#10143=FACE_OUTER_BOUND ( 'NONE', #86244, .T. ) ;
#10144=DIRECTION ( 'NONE',  ( 0.000000000000000000, 0.000000000000000000, 1.000000000000000000 ) ) ;
#10145=CARTESIAN_POINT ( 'NONE',  ( -3.350000000000032507, 2.500000000000000000, -6.495190528383302464 ) ) ;
#10146=DIRECTION ( 'NONE',  ( 0.000000000000000000, -0.9999939076577903929, 0.003490651415223739937 ) ) ;
#10147=AXIS2_PLACEMENT_3D ( 'NONE', #87874, #78745, #27047 ) ;
#10148=CARTESIAN_POINT ( 'NONE',  ( -8.150000000000014566, 12.50000000000000000, -6.148780366869520897 ) ) ;
#10149=CARTESIAN_POINT ( 'NONE',  ( 7.299999999999924327, 12.50000000000000000, 0.4115034346978109769 ) ) ;
#10150=DIRECTION ( 'NONE',  ( 0.000000000000000000, -0.000000000000000000, 1.000000000000000000 ) ) ;
#10151=CIRCLE ( 'NONE', #123022, 0.06509327318403745899 ) ;
#10153=ORIENTED_EDGE ( 'NONE', *, *, #31291, .T. ) ;
#10154=ORIENTED_EDGE ( 'NONE', *, *, #67446, .T. ) ;
#10155=CIRCLE ( 'NONE', #52020, 0.06509327318403745899 ) ;
#10156=ORIENTED_EDGE ( 'NONE', *, *, #11879, .T. ) ;
#10157=ORIENTED_EDGE ( 'NONE', *, *, #110114, .T. ) ;
#10158=CARTESIAN_POINT ( 'NONE',  ( -11.05000000000000249, 12.50000000000000000, -6.213873640053560798 ) ) ;
#10159=DIRECTION ( 'NONE',  ( -0.000000000000000000, 1.000000000000000000, -0.000000000000000000 ) ) ;
#10160=ORIENTED_EDGE ( 'NONE', *, *, #73767, .F. ) ;
#10161=FACE_BOUND ( 'NONE', #92678, .T. ) ;
#10162=PLANE ( 'NONE',  #68802 ) ;
#10163=AXIS2_PLACEMENT_3D ( 'NONE', #117876, #56380, #86487 ) ;
#10164=AXIS2_PLACEMENT_3D ( 'NONE', #45159, #26154, #14374 ) ;
#10165=EDGE_CURVE ( 'NONE', #106006, #40443, #41982, .T. ) ;
#10166=AXIS2_PLACEMENT_3D ( 'NONE', #94958, #24918, #95594 ) ;
#10167=VECTOR ( 'NONE', #120613, 1000.000000000000000 ) ;
#10168=CARTESIAN_POINT ( 'NONE',  ( 3.349999999999943689, 2.500000000000000000, 1.372243186433545370 ) ) ;
#10169=ADVANCED_FACE ( 'NONE', ( #122731 ), #2334, .T. ) ;
#10170=DIRECTION ( 'NONE',  ( 0.000000000000000000, 0.000000000000000000, 1.000000000000000000 ) ) ;
#10171=CARTESIAN_POINT ( 'NONE',  ( -3.350000000000028955, 12.50000000000000000, 5.802370205355744659 ) ) ;
#10172=FACE_OUTER_BOUND ( 'NONE', #24662, .T. ) ;
#10173=DIRECTION ( 'NONE',  ( 0.000000000000000000, -0.9999939076577903929, 0.003490651415223739937 ) ) ;
#10174=VERTEX_POINT ( 'NONE', #45478 ) ;
#10175=AXIS2_PLACEMENT_3D ( 'NONE', #52148, #81598, #11564 ) ;
#10176=ADVANCED_FACE ( 'NONE', ( #83466 ), #74922, .T. ) ;
#10177=ORIENTED_EDGE ( 'NONE', *, *, #35053, .F. ) ;
#10178=AXIS2_PLACEMENT_3D ( 'NONE', #66735, #5240, #25514 ) ;
#10179=ORIENTED_EDGE ( 'NONE', *, *, #60516, .F. ) ;
#10180=ORIENTED_EDGE ( 'NONE', *, *, #55762, .T. ) ;
#10181=VERTEX_POINT ( 'NONE', #14683 ) ;
#10182=VERTEX_POINT ( 'NONE', #53992 ) ;
#10183=CARTESIAN_POINT ( 'NONE',  ( -0.8500000000000395017, 2.500000000000000000, 6.495190528383297135 ) ) ;
#10184=DIRECTION ( 'NONE',  ( 0.000000000000000000, 1.000000000000000000, 0.000000000000000000 ) ) ;
#10185=EDGE_LOOP ( 'NONE', ( #50471, #33302 ) ) ;
#10186=CARTESIAN_POINT ( 'NONE',  ( -13.74999999999995381, 2.500000000000000000, 2.065063509461101621 ) ) ;
#10187=CIRCLE ( 'NONE', #47844, 0.1000000000000000472 ) ;
#10188=CARTESIAN_POINT ( 'NONE',  ( 7.049999999999926992, 12.50000000000000000, 2.099970236277060032 ) ) ;
#10190=CARTESIAN_POINT ( 'NONE',  ( 11.44999999999990514, 2.500000000000000000, -6.048780366869526581 ) ) ;
#10191=FACE_OUTER_BOUND ( 'NONE', #14531, .T. ) ;
#10192=AXIS2_PLACEMENT_3D ( 'NONE', #109402, #119870, #31496 ) ;
#10193=ORIENTED_EDGE ( 'NONE', *, *, #50639, .F. ) ;
#10194=DIRECTION ( 'NONE',  ( 0.000000000000000000, 0.000000000000000000, 1.000000000000000000 ) ) ;
#10195=ORIENTED_EDGE ( 'NONE', *, *, #89306, .F. ) ;
#10196=EDGE_LOOP ( 'NONE', ( #18457, #105235 ) ) ;
#10198=DIRECTION ( 'NONE',  ( 0.000000000000000000, 1.000000000000000000, 0.000000000000000000 ) ) ;
#10199=DIRECTION ( 'NONE',  ( 0.000000000000000000, 0.000000000000000000, 1.000000000000000000 ) ) ;
#10200=CARTESIAN_POINT ( 'NONE',  ( 0.8499999999999553468, 2.500000000000000000, 2.165063509461097713 ) ) ;
#10201=VERTEX_POINT ( 'NONE', #125306 ) ;
#10202=AXIS2_PLACEMENT_3D ( 'NONE', #48053, #126614, #76223 ) ;
#10203=ORIENTED_EDGE ( 'NONE', *, *, #83296, .T. ) ;
#10205=DIRECTION ( 'NONE',  ( 0.000000000000000000, 1.000000000000000000, 0.000000000000000000 ) ) ;
#10206=AXIS2_PLACEMENT_3D ( 'NONE', #3978, #83827, #105418 ) ;
#10207=DIRECTION ( 'NONE',  ( 0.000000000000000000, 0.000000000000000000, -1.000000000000000000 ) ) ;
#10208=CARTESIAN_POINT ( 'NONE',  ( -10.00000000000000355, 12.50000000000000000, -0.7579135962115916003 ) ) ;
#10209=CARTESIAN_POINT ( 'NONE',  ( 8.299999999999922551, 2.500000000000000000, -0.1000000000000023925 ) ) ;
#10210=ORIENTED_EDGE ( 'NONE', *, *, #38957, .T. ) ;
#10211=LINE ( 'NONE', #72363, #85768 ) ;
#10212=AXIS2_PLACEMENT_3D ( 'NONE', #25806, #33694, #84071 ) ;
#10213=VERTEX_POINT ( 'NONE', #85380 ) ;
#10214=FACE_OUTER_BOUND ( 'NONE', #89986, .T. ) ;
#10215=ORIENTED_EDGE ( 'NONE', *, *, #12098, .T. ) ;
#10216=CARTESIAN_POINT ( 'NONE',  ( -9.600000000000008527, 2.500000000000000000, -4.330127018922197202 ) ) ;
#10217=AXIS2_PLACEMENT_3D ( 'NONE', #2023, #101529, #32161 ) ;
#10218=AXIS2_PLACEMENT_3D ( 'NONE', #60217, #54243, #32696 ) ;
#10219=CARTESIAN_POINT ( 'NONE',  ( 15.79999999999989058, 2.500000000000000000, -2.385244779468109755E-15 ) ) ;
#10220=DIRECTION ( 'NONE',  ( 0.000000000000000000, 1.000000000000000000, 0.000000000000000000 ) ) ;
#10221=EDGE_CURVE ( 'NONE', #14604, #92039, #67169, .T. ) ;
#10222=ADVANCED_FACE ( 'NONE', ( #35644 ), #33750, .T. ) ;
#10223=LINE ( 'NONE', #50159, #114883 ) ;
#10224=VERTEX_POINT ( 'NONE', #124012 ) ;
#10225=CARTESIAN_POINT ( 'NONE',  ( 17.49862860983209245, -2.500000000000000000, 4.081131818001135336 ) ) ;
#10226=VECTOR ( 'NONE', #26008, 1000.000000000000000 ) ;
#10227=CIRCLE ( 'NONE', #1796, 0.06509327318403745899 ) ;
#10228=DIRECTION ( 'NONE',  ( -0.000000000000000000, -1.000000000000000000, -0.000000000000000000 ) ) ;
#10229=ORIENTED_EDGE ( 'NONE', *, *, #164, .T. ) ;
#10230=EDGE_LOOP ( 'NONE', ( #87209, #36426 ) ) ;
#10231=ADVANCED_FACE ( 'NONE', ( #113550 ), #95851, .T. ) ;
#10232=ORIENTED_EDGE ( 'NONE', *, *, #5784, .F. ) ;
#10233=DIRECTION ( 'NONE',  ( 0.000000000000000000, 0.000000000000000000, -1.000000000000000000 ) ) ;
#10234=DIRECTION ( 'NONE',  ( 0.000000000000000000, -0.9999939076577903929, 0.003490651415223739937 ) ) ;
#10235=FACE_OUTER_BOUND ( 'NONE', #72739, .T. ) ;
#10236=DIRECTION ( 'NONE',  ( 0.000000000000000000, 0.000000000000000000, 1.000000000000000000 ) ) ;
#10237=CARTESIAN_POINT ( 'NONE',  ( -12.89999999999999147, 2.500000000000000000, -0.7928203230275501223 ) ) ;
#10238=CARTESIAN_POINT ( 'NONE',  ( -6.650000000000019007, 2.500000000000000000, -5.802370205355749988 ) ) ;
#10239=DIRECTION ( 'NONE',  ( 0.000000000000000000, 0.000000000000000000, -1.000000000000000000 ) ) ;
#10240=CARTESIAN_POINT ( 'NONE',  ( -0.6500000000000403233, 2.500000000000000000, 6.248780366869520542 ) ) ;
#10242=AXIS2_PLACEMENT_3D ( 'NONE', #8370, #48309, #28679 ) ;
#10243=CONICAL_SURFACE ( 'NONE', #93863, 0.1000000000000002554, 0.003490658503988666988 ) ;
#10244=AXIS2_PLACEMENT_3D ( 'NONE', #79779, #30047, #109892 ) ;
#10245=VERTEX_POINT ( 'NONE', #116122 ) ;
#10246=DIRECTION ( 'NONE',  ( 0.000000000000000000, 1.000000000000000000, 0.000000000000000000 ) ) ;
#10247=DIRECTION ( 'NONE',  ( 0.000000000000000000, -0.9999939076577903929, 0.003490651415223739937 ) ) ;
#10248=CARTESIAN_POINT ( 'NONE',  ( 12.69999999999989981, 2.500000000000000000, -0.3464101615137783474 ) ) ;
#10249=DIRECTION ( 'NONE',  ( -0.000000000000000000, 1.000000000000000000, -0.000000000000000000 ) ) ;
#10250=CARTESIAN_POINT ( 'NONE',  ( 6.849999999999930367, 12.50000000000000000, -6.841600689897078702 ) ) ;
#10251=VECTOR ( 'NONE', #125345, 1000.000000000000000 ) ;
#10252=ORIENTED_EDGE ( 'NONE', *, *, #10121, .F. ) ;
#10253=CIRCLE ( 'NONE', #116842, 0.06509327318403745899 ) ;
#10254=DIRECTION ( 'NONE',  ( 0.000000000000000000, 1.000000000000000000, 0.000000000000000000 ) ) ;
#10255=EDGE_CURVE ( 'NONE', #56832, #30668, #65028, .T. ) ;
#10256=CIRCLE ( 'NONE', #77063, 0.06509327318403745899 ) ;
#10257=DIRECTION ( 'NONE',  ( 0.000000000000000000, 0.000000000000000000, 1.000000000000000000 ) ) ;
#10258=DIRECTION ( 'NONE',  ( 0.000000000000000000, -0.000000000000000000, 1.000000000000000000 ) ) ;
#10259=EDGE_LOOP ( 'NONE', ( #33853, #41497, #85202, #50407 ) ) ;
#10260=EDGE_CURVE ( 'NONE', #89429, #125138, #34367, .T. ) ;
#10261=AXIS2_PLACEMENT_3D ( 'NONE', #113479, #13334, #55219 ) ;
#10262=EDGE_CURVE ( 'NONE', #72798, #88688, #79723, .T. ) ;
#10263=EDGE_LOOP ( 'NONE', ( #117870, #106023 ) ) ;
#10264=LINE ( 'NONE', #2344, #86471 ) ;
#10265=AXIS2_PLACEMENT_3D ( 'NONE', #61456, #71919, #91544 ) ;
#10266=ORIENTED_EDGE ( 'NONE', *, *, #114870, .F. ) ;
#10267=ORIENTED_EDGE ( 'NONE', *, *, #48638, .F. ) ;
#10268=DIRECTION ( 'NONE',  ( 0.000000000000000000, 0.000000000000000000, 1.000000000000000000 ) ) ;
#10270=EDGE_CURVE ( 'NONE', #60027, #51534, #125932, .T. ) ;
#10271=ADVANCED_FACE ( 'NONE', ( #85999 ), #44164, .T. ) ;
#10272=DIRECTION ( 'NONE',  ( 0.000000000000000000, 0.000000000000000000, -1.000000000000000000 ) ) ;
#10273=DIRECTION ( 'NONE',  ( 0.000000000000000000, 0.000000000000000000, 1.000000000000000000 ) ) ;
#10274=AXIS2_PLACEMENT_3D ( 'NONE', #78784, #38204, #37564 ) ;
#10275=ORIENTED_EDGE ( 'NONE', *, *, #80598, .F. ) ;
#10276=ADVANCED_FACE ( 'NONE', ( #74281 ), #102694, .T. ) ;
#10278=ORIENTED_EDGE ( 'NONE', *, *, #25010, .T. ) ;
#10279=VECTOR ( 'NONE', #38211, 1000.000000000000000 ) ;
#10280=FACE_OUTER_BOUND ( 'NONE', #58839, .T. ) ;
#10281=DIRECTION ( 'NONE',  ( 0.000000000000000000, -0.000000000000000000, 1.000000000000000000 ) ) ;
#10282=DIRECTION ( 'NONE',  ( -0.000000000000000000, -1.000000000000000000, -0.000000000000000000 ) ) ;
#10283=EDGE_CURVE ( 'NONE', #92342, #26773, #16621, .T. ) ;
#10284=EDGE_LOOP ( 'NONE', ( #25411, #70188 ) ) ;
#10285=ORIENTED_EDGE ( 'NONE', *, *, #25745, .F. ) ;
#10286=EDGE_LOOP ( 'NONE', ( #28362, #66749 ) ) ;
#10287=EDGE_LOOP ( 'NONE', ( #76051, #104201, #24533, #127231 ) ) ;
#10288=ORIENTED_EDGE ( 'NONE', *, *, #51644, .F. ) ;
#10289=DIRECTION ( 'NONE',  ( -0.000000000000000000, 1.000000000000000000, -0.000000000000000000 ) ) ;
#10290=CARTESIAN_POINT ( 'NONE',  ( 10.89704209861837647, 2.499999999999872990, 8.980393935569876973 ) ) ;
#10291=DIRECTION ( 'NONE',  ( 0.000000000000000000, -0.9999939076577903929, 0.003490651415223739937 ) ) ;
#10292=FACE_BOUND ( 'NONE', #8559, .T. ) ;
#10293=PLANE ( 'NONE',  #30617 ) ;
#10294=CARTESIAN_POINT ( 'NONE',  ( -9.550000000000002487, 2.500000000000000000, 6.395190528383296602 ) ) ;
#10295=CIRCLE ( 'NONE', #35433, 0.06509327318403745899 ) ;
#10296=CARTESIAN_POINT ( 'NONE',  ( -5.600000000000020073, 2.500000000000000000, -0.4464101615137782142 ) ) ;
#10297=DIRECTION ( 'NONE',  ( 0.000000000000000000, 0.000000000000000000, 1.000000000000000000 ) ) ;
#10298=AXIS2_PLACEMENT_3D ( 'NONE', #604, #116194, #55357 ) ;
#10299=DIRECTION ( 'NONE',  ( 0.000000000000000000, -0.9999939076577903929, 0.003490651415223739937 ) ) ;
#10300=DIRECTION ( 'NONE',  ( 0.000000000000000000, -0.9999939076577903929, 0.003490651415223739937 ) ) ;
#10301=CIRCLE ( 'NONE', #18700, 0.1000000000000002554 ) ;
#10302=CARTESIAN_POINT ( 'NONE',  ( -3.100000000000028511, 2.500000000000000000, -0.3464101615137782364 ) ) ;
#10303=DIRECTION ( 'NONE',  ( 0.000000000000000000, -0.9999939076577903929, 0.003490651415223739937 ) ) ;
#10304=VECTOR ( 'NONE', #48241, 1000.000000000000000 ) ;
#10305=CONICAL_SURFACE ( 'NONE', #125323, 0.09999999999999999167, 0.003490658503988666988 ) ;
#10306=ORIENTED_EDGE ( 'NONE', *, *, #129115, .T. ) ;
#10307=ORIENTED_EDGE ( 'NONE', *, *, #46934, .F. ) ;
#10309=ORIENTED_EDGE ( 'NONE', *, *, #122529, .F. ) ;
#10310=CARTESIAN_POINT ( 'NONE',  ( -3.350000000000029399, 2.500000000000000000, 6.495190528383297135 ) ) ;
#10311=DIRECTION ( 'NONE',  ( -4.274815082592931898E-19, -0.9999939076577903929, -0.003490651415223739937 ) ) ;
#10312=FACE_BOUND ( 'NONE', #115454, .T. ) ;
#10313=DIRECTION ( 'NONE',  ( 0.000000000000000000, -0.9999939076577903929, 0.003490651415223739937 ) ) ;
#10314=CIRCLE ( 'NONE', #8153, 0.1000000000000002554 ) ;
#10315=CIRCLE ( 'NONE', #6086, 0.06509327318403745899 ) ;
#10316=EDGE_CURVE ( 'NONE', #29957, #82736, #33702, .T. ) ;
#10317=ORIENTED_EDGE ( 'NONE', *, *, #13465, .T. ) ;
#10318=DIRECTION ( 'NONE',  ( -0.000000000000000000, -1.000000000000000000, -0.000000000000000000 ) ) ;
#10319=DIRECTION ( 'NONE',  ( 0.000000000000000000, 1.000000000000000000, 0.000000000000000000 ) ) ;
#10320=LINE ( 'NONE', #20145, #122079 ) ;
#10321=CARTESIAN_POINT ( 'NONE',  ( 9.349999999999916156, 2.500000000000000000, 6.741600689897071952 ) ) ;
#10322=ORIENTED_EDGE ( 'NONE', *, *, #100961, .T. ) ;
#10323=CARTESIAN_POINT ( 'NONE',  ( 14.34999999999989306, 12.50000000000000000, -2.511473670974877948 ) ) ;
#10324=EDGE_CURVE ( 'NONE', #31484, #6262, #12799, .T. ) ;
#10325=ORIENTED_EDGE ( 'NONE', *, *, #42018, .F. ) ;
#10326=ORIENTED_EDGE ( 'NONE', *, *, #49141, .T. ) ;
#10327=CONICAL_SURFACE ( 'NONE', #83505, 0.09999999999999982514, 0.003490658503988666988 ) ;
#10330=ORIENTED_EDGE ( 'NONE', *, *, #64792, .T. ) ;
#10331=AXIS2_PLACEMENT_3D ( 'NONE', #5089, #103955, #36516 ) ;
#10332=DIRECTION ( 'NONE',  ( -0.000000000000000000, -1.000000000000000000, -0.000000000000000000 ) ) ;
#10333=CIRCLE ( 'NONE', #93865, 0.06509327318403745899 ) ;
#10334=DIRECTION ( 'NONE',  ( -0.000000000000000000, -1.000000000000000000, -0.000000000000000000 ) ) ;
#10335=DIRECTION ( 'NONE',  ( 0.000000000000000000, 0.000000000000000000, 1.000000000000000000 ) ) ;
#10336=ORIENTED_EDGE ( 'NONE', *, *, #112879, .F. ) ;
#10337=LINE ( 'NONE', #41754, #105888 ) ;
#10338=ORIENTED_EDGE ( 'NONE', *, *, #23260, .F. ) ;
#10339=FACE_OUTER_BOUND ( 'NONE', #107515, .T. ) ;
#10340=VECTOR ( 'NONE', #97313, 1000.000000000000000 ) ;
#10341=VERTEX_POINT ( 'NONE', #97134 ) ;
#10343=ORIENTED_EDGE ( 'NONE', *, *, #115651, .T. ) ;
#10344=DIRECTION ( 'NONE',  ( 0.000000000000000000, 0.000000000000000000, -1.000000000000000000 ) ) ;
#10345=CARTESIAN_POINT ( 'NONE',  ( -6.850000000000013856, 2.500000000000000000, 2.511473670974873507 ) ) ;
#10346=DIRECTION ( 'NONE',  ( 0.000000000000000000, -0.000000000000000000, 1.000000000000000000 ) ) ;
#10347=DIRECTION ( 'NONE',  ( 0.000000000000000000, 0.000000000000000000, 1.000000000000000000 ) ) ;
#10348=CARTESIAN_POINT ( 'NONE',  ( -10.40000000000000213, 2.500000000000000000, -4.922947341949749145 ) ) ;
#10349=ORIENTED_EDGE ( 'NONE', *, *, #84997, .F. ) ;
#10350=ORIENTED_EDGE ( 'NONE', *, *, #97974, .T. ) ;
#10351=AXIS2_PLACEMENT_3D ( 'NONE', #30401, #70306, #10703 ) ;
#10352=EDGE_CURVE ( 'NONE', #56130, #93998, #88008, .T. ) ;
#10353=ORIENTED_EDGE ( 'NONE', *, *, #120614, .T. ) ;
#10354=DIRECTION ( 'NONE',  ( -0.000000000000000000, -1.000000000000000000, -0.000000000000000000 ) ) ;
#10355=CIRCLE ( 'NONE', #71001, 0.1000000000000002554 ) ;
#10356=CARTESIAN_POINT ( 'NONE',  ( 4.349999999999940137, 12.50000000000000000, -2.511473670974877948 ) ) ;
#10357=CARTESIAN_POINT ( 'NONE',  ( 11.84999999999990727, 12.50000000000000000, 6.841600689897072485 ) ) ;
#10358=ORIENTED_EDGE ( 'NONE', *, *, #53673, .F. ) ;
#10359=ORIENTED_EDGE ( 'NONE', *, *, #53160, .T. ) ;
#10360=ORIENTED_EDGE ( 'NONE', *, *, #114124, .T. ) ;
#10361=CARTESIAN_POINT ( 'NONE',  ( 8.549999999999924327, 2.500000000000000000, -6.841600689897077814 ) ) ;
#10362=ORIENTED_EDGE ( 'NONE', *, *, #76940, .F. ) ;
#10363=CARTESIAN_POINT ( 'NONE',  ( 11.44999999999990870, 12.50000000000000000, -1.883746621131363597 ) ) ;
#10364=EDGE_CURVE ( 'NONE', #109058, #33086, #14934, .T. ) ;
#10366=CARTESIAN_POINT ( 'NONE',  ( 6.649999999999931966, 12.50000000000000000, -5.802370205355749988 ) ) ;
#10367=CARTESIAN_POINT ( 'NONE',  ( 97.50000000000000000, 0.000000000000000000, 0.000000000000000000 ) ) ;
#10368=DIRECTION ( 'NONE',  ( -4.274815082592931898E-19, -0.9999939076577903929, -0.003490651415223739937 ) ) ;
#10369=CARTESIAN_POINT ( 'NONE',  ( -8.950000000000009948, 2.500000000000000000, -1.718653347947326049 ) ) ;
#10370=AXIS2_PLACEMENT_3D ( 'NONE', #110799, #49978, #89869 ) ;
#10371=CARTESIAN_POINT ( 'NONE',  ( -8.100000000000010303, 2.500000000000000000, 4.083716857408421497 ) ) ;
#10372=ADVANCED_FACE ( 'NONE', ( #129209 ), #59158, .T. ) ;
#10373=EDGE_CURVE ( 'NONE', #3125, #55337, #108241, .T. ) ;
#10374=CARTESIAN_POINT ( 'NONE',  ( 12.04999999999990479, 2.500000000000000000, 2.265063509461097357 ) ) ;
#10375=VERTEX_POINT ( 'NONE', #18576 ) ;
#10376=EDGE_LOOP ( 'NONE', ( #91942, #128514 ) ) ;
#10377=CARTESIAN_POINT ( 'NONE',  ( 11.04999999999990656, 12.50000000000000000, -6.213873640053564351 ) ) ;
#10378=ADVANCED_FACE ( 'NONE', ( #118704 ), #42083, .T. ) ;
#10379=EDGE_LOOP ( 'NONE', ( #94276, #128373, #80964, #94938 ) ) ;
#10380=EDGE_LOOP ( 'NONE', ( #5509, #123472, #55811, #92993 ) ) ;
#10381=EDGE_CURVE ( 'NONE', #2782, #17144, #29551, .T. ) ;
#10383=FACE_OUTER_BOUND ( 'NONE', #45505, .T. ) ;
#10384=DIRECTION ( 'NONE',  ( 0.000000000000000000, 0.000000000000000000, 1.000000000000000000 ) ) ;
#10385=FACE_OUTER_BOUND ( 'NONE', #62794, .T. ) ;
#10386=CARTESIAN_POINT ( 'NONE',  ( 7.499999999999927169, 2.500000000000000000, -5.022947341949754119 ) ) ;
#10387=DIRECTION ( 'NONE',  ( -4.274815082592931898E-19, -0.9999939076577903929, -0.003490651415223739937 ) ) ;
#10388=DIRECTION ( 'NONE',  ( 0.000000000000000000, -0.000000000000000000, 1.000000000000000000 ) ) ;
#10389=CIRCLE ( 'NONE', #129553, 0.1000000000000002554 ) ;
#10390=DIRECTION ( 'NONE',  ( 0.000000000000000000, 1.000000000000000000, 0.000000000000000000 ) ) ;
#10391=VERTEX_POINT ( 'NONE', #49352 ) ;
#10392=AXIS2_PLACEMENT_3D ( 'NONE', #73034, #5563, #92677 ) ;
#10393=EDGE_LOOP ( 'NONE', ( #28580, #116103 ) ) ;
#10394=AXIS2_PLACEMENT_3D ( 'NONE', #126564, #38179, #95805 ) ;
#10395=VERTEX_POINT ( 'NONE', #97781 ) ;
#10396=ORIENTED_EDGE ( 'NONE', *, *, #68744, .F. ) ;
#10397=DIRECTION ( 'NONE',  ( 0.000000000000000000, -0.9999939076577903929, 0.003490651415223739937 ) ) ;
#10398=CARTESIAN_POINT ( 'NONE',  ( -9.800000000000006040, 12.50000000000000000, -4.676537180435974328 ) ) ;
#10399=AXIS2_PLACEMENT_3D ( 'NONE', #110218, #9439, #19910 ) ;
#10400=CIRCLE ( 'NONE', #37611, 0.1000000000000002554 ) ;
#10401=EDGE_LOOP ( 'NONE', ( #106524, #16514 ) ) ;
#10402=DIRECTION ( 'NONE',  ( -4.274815082592931898E-19, -0.9999939076577903929, -0.003490651415223739937 ) ) ;
#10403=EDGE_CURVE ( 'NONE', #99398, #104575, #27465, .T. ) ;
#10405=CARTESIAN_POINT ( 'NONE',  ( -4.200000000000029488, 2.500000000000000000, -4.230127018922201998 ) ) ;
#10406=DIRECTION ( 'NONE',  ( 0.000000000000000000, 1.000000000000000000, 0.000000000000000000 ) ) ;
#10408=DIRECTION ( 'NONE',  ( 0.000000000000000000, 0.000000000000000000, -1.000000000000000000 ) ) ;
#10409=EDGE_CURVE ( 'NONE', #78466, #33313, #16977, .T. ) ;
#10410=CARTESIAN_POINT ( 'NONE',  ( -3.100000000000028511, 2.500000000000000000, 0.3464101615137736845 ) ) ;
#10411=ORIENTED_EDGE ( 'NONE', *, *, #1075, .F. ) ;
#10412=ORIENTED_EDGE ( 'NONE', *, *, #42994, .F. ) ;
#10413=ORIENTED_EDGE ( 'NONE', *, *, #90137, .T. ) ;
#10415=CARTESIAN_POINT ( 'NONE',  ( 12.69999999999989981, 12.50000000000000000, -0.2813168883297409439 ) ) ;
#10416=EDGE_CURVE ( 'NONE', #2020, #74876, #58799, .T. ) ;
#10417=ADVANCED_FACE ( 'NONE', ( #27108 ), #47400, .T. ) ;
#10418=EDGE_CURVE ( 'NONE', #96223, #11828, #119346, .T. ) ;
#10419=LINE ( 'NONE', #50349, #115697 ) ;
#10420=CARTESIAN_POINT ( 'NONE',  ( 9.799999999999915445, 2.500000000000000000, 3.983716857408420964 ) ) ;
#10421=CONICAL_SURFACE ( 'NONE', #117007, 0.1000000000000002554, 0.003490658503988666988 ) ;
#10422=ADVANCED_FACE ( 'NONE', ( #69601 ), #100634, .T. ) ;
#10423=DIRECTION ( 'NONE',  ( -4.274815082592931898E-19, -0.9999939076577903929, -0.003490651415223739937 ) ) ;
#10424=ORIENTED_EDGE ( 'NONE', *, *, #38710, .F. ) ;
#10425=CARTESIAN_POINT ( 'NONE',  ( -10.85000000000000142, 2.500000000000000000, -2.165063509461097713 ) ) ;
#10426=DIRECTION ( 'NONE',  ( 0.000000000000000000, -0.000000000000000000, 1.000000000000000000 ) ) ;
#10427=DIRECTION ( 'NONE',  ( 0.000000000000000000, -0.000000000000000000, 1.000000000000000000 ) ) ;
#10428=CARTESIAN_POINT ( 'NONE',  ( -10.45000000000000462, 12.50000000000000000, -2.099970236277060476 ) ) ;
#10430=ADVANCED_FACE ( 'NONE', ( #87936 ), #14849, .T. ) ;
#10431=ORIENTED_EDGE ( 'NONE', *, *, #93477, .T. ) ;
#10432=EDGE_CURVE ( 'NONE', #26094, #49778, #56711, .T. ) ;
#10433=CARTESIAN_POINT ( 'NONE',  ( 11.24999999999990585, 12.50000000000000000, 2.857883832488649301 ) ) ;
#10434=ORIENTED_EDGE ( 'NONE', *, *, #125767, .F. ) ;
#10435=ORIENTED_EDGE ( 'NONE', *, *, #88989, .T. ) ;
#10436=DIRECTION ( 'NONE',  ( 0.000000000000000000, 1.000000000000000000, 0.000000000000000000 ) ) ;
#10437=CARTESIAN_POINT ( 'NONE',  ( 2.099999999999947686, 2.500000000000000000, 4.922947341949748257 ) ) ;
#10438=FACE_BOUND ( 'NONE', #97319, .T. ) ;
#10440=PLANE ( 'NONE',  #57609 ) ;
#10441=CARTESIAN_POINT ( 'NONE',  ( 8.149999999999920419, 2.500000000000000000, -1.818653347947325916 ) ) ;
#10442=DIRECTION ( 'NONE',  ( 0.000000000000000000, 0.000000000000000000, 1.000000000000000000 ) ) ;
#10443=CONICAL_SURFACE ( 'NONE', #123310, 0.09999999999999982514, 0.003490658503988666988 ) ;
#10444=CIRCLE ( 'NONE', #2122, 0.1000000000000000472 ) ;
#10445=DIRECTION ( 'NONE',  ( 0.000000000000000000, 1.000000000000000000, 0.000000000000000000 ) ) ;
#10446=CARTESIAN_POINT ( 'NONE',  ( -12.89999999999999147, 2.500000000000000000, 5.022947341949748790 ) ) ;
#10447=DIRECTION ( 'NONE',  ( 0.000000000000000000, 0.000000000000000000, 1.000000000000000000 ) ) ;
#10448=CARTESIAN_POINT ( 'NONE',  ( -11.64999999999999680, 2.500000000000000000, 7.188010851410848723 ) ) ;
#10449=ORIENTED_EDGE ( 'NONE', *, *, #78188, .F. ) ;
#10450=CONICAL_SURFACE ( 'NONE', #33457, 0.1000000000000002554, 0.003490658503988666988 ) ;
#10451=DIRECTION ( 'NONE',  ( 0.000000000000000000, 0.000000000000000000, 1.000000000000000000 ) ) ;
#10452=DIRECTION ( 'NONE',  ( 0.000000000000000000, -0.9999939076577903929, 0.003490651415223739937 ) ) ;
#10453=CIRCLE ( 'NONE', #35602, 0.09999999999999982514 ) ;
#10454=ORIENTED_EDGE ( 'NONE', *, *, #28755, .T. ) ;
#10455=ORIENTED_EDGE ( 'NONE', *, *, #64339, .F. ) ;
#10457=CARTESIAN_POINT ( 'NONE',  ( -11.24999999999996270, 12.50000000000000000, 6.495190528383297135 ) ) ;
#10458=FACE_BOUND ( 'NONE', #81099, .T. ) ;
#10459=CARTESIAN_POINT ( 'NONE',  ( 2.699999999999944666, 2.500000000000000000, 4.576537180435972019 ) ) ;
#10460=DIRECTION ( 'NONE',  ( -0.000000000000000000, -1.000000000000000000, -0.000000000000000000 ) ) ;
#10461=ADVANCED_FACE ( 'NONE', ( #128562 ), #81766, .T. ) ;
#10462=ORIENTED_EDGE ( 'NONE', *, *, #112154, .F. ) ;
#10463=DIRECTION ( 'NONE',  ( 0.000000000000000000, 1.000000000000000000, 0.000000000000000000 ) ) ;
#10464=DIRECTION ( 'NONE',  ( 0.000000000000000000, 0.000000000000000000, -1.000000000000000000 ) ) ;
#10466=CARTESIAN_POINT ( 'NONE',  ( -12.49999999999999467, 2.500000000000000000, 0.5928203230275536084 ) ) ;
#10468=EDGE_CURVE ( 'NONE', #60755, #88674, #106938, .T. ) ;
#10469=CARTESIAN_POINT ( 'NONE',  ( 12.49999999999990585, 12.50000000000000000, 3.702399969078682407 ) ) ;
#10470=CARTESIAN_POINT ( 'NONE',  ( 2.049999999999950084, 2.500000000000000000, 2.165063509461097713 ) ) ;
#10471=VERTEX_POINT ( 'NONE', #28405 ) ;
#10472=DIRECTION ( 'NONE',  ( -0.000000000000000000, 1.000000000000000000, -0.000000000000000000 ) ) ;
#10473=AXIS2_PLACEMENT_3D ( 'NONE', #91236, #30408, #41516 ) ;
#10474=CIRCLE ( 'NONE', #123359, 0.06509327318403745899 ) ;
#10475=DIRECTION ( 'NONE',  ( 0.000000000000000000, 1.000000000000000000, 0.000000000000000000 ) ) ;
#10476=DIRECTION ( 'NONE',  ( 0.000000000000000000, -0.000000000000000000, 1.000000000000000000 ) ) ;
#10477=CARTESIAN_POINT ( 'NONE',  ( 1.249999999999988454, 2.500000000000000000, -2.165063509461101710 ) ) ;
#10479=EDGE_LOOP ( 'NONE', ( #38773, #96171, #50215, #74747 ) ) ;
#10480=CARTESIAN_POINT ( 'NONE',  ( -8.750000000000008882, 12.50000000000000000, -2.857883832488653741 ) ) ;
#10481=ORIENTED_EDGE ( 'NONE', *, *, #110242, .T. ) ;
#10482=DIRECTION ( 'NONE',  ( 0.000000000000000000, 1.000000000000000000, 0.000000000000000000 ) ) ;
#10483=AXIS2_PLACEMENT_3D ( 'NONE', #47929, #28280, #96351 ) ;
#10484=DIRECTION ( 'NONE',  ( 0.000000000000000000, 0.000000000000000000, 1.000000000000000000 ) ) ;
#10485=CARTESIAN_POINT ( 'NONE',  ( 10.84999999999990905, 12.50000000000000000, 1.537336459617582918 ) ) ;
#10486=EDGE_LOOP ( 'NONE', ( #93915, #95916, #77096, #37661 ) ) ;
#10487=DIRECTION ( 'NONE',  ( 0.000000000000000000, 1.000000000000000000, 0.000000000000000000 ) ) ;
#10488=CARTESIAN_POINT ( 'NONE',  ( -5.450000000000023270, 2.500000000000000000, -6.495190528383302464 ) ) ;
#10489=DIRECTION ( 'NONE',  ( 0.000000000000000000, 0.000000000000000000, 1.000000000000000000 ) ) ;
#10490=DIRECTION ( 'NONE',  ( 0.000000000000000000, -0.000000000000000000, 1.000000000000000000 ) ) ;
#10491=DIRECTION ( 'NONE',  ( 0.000000000000000000, 1.000000000000000000, 0.000000000000000000 ) ) ;
#10492=DIRECTION ( 'NONE',  ( 0.000000000000000000, 0.000000000000000000, 1.000000000000000000 ) ) ;
#10493=ORIENTED_EDGE ( 'NONE', *, *, #124185, .F. ) ;
#10494=ORIENTED_EDGE ( 'NONE', *, *, #83444, .F. ) ;
#10495=DIRECTION ( 'NONE',  ( 0.000000000000000000, 1.000000000000000000, 0.000000000000000000 ) ) ;
#10496=VERTEX_POINT ( 'NONE', #32935 ) ;
#10497=CARTESIAN_POINT ( 'NONE',  ( 2.099999999999950351, 2.500000000000000000, -4.330127018922201643 ) ) ;
#10498=ORIENTED_EDGE ( 'NONE', *, *, #60829, .T. ) ;
#10499=ORIENTED_EDGE ( 'NONE', *, *, #31682, .T. ) ;
#10500=VERTEX_POINT ( 'NONE', #49995 ) ;
#10501=CARTESIAN_POINT ( 'NONE',  ( 17.50000000000000000, 0.8333333333333378112, -3.999999999999996447 ) ) ;
#10502=AXIS2_PLACEMENT_3D ( 'NONE', #30181, #121756, #62218 ) ;
#10503=DIRECTION ( 'NONE',  ( 0.000000000000000000, 1.000000000000000000, 0.000000000000000000 ) ) ;
#10504=EDGE_CURVE ( 'NONE', #50078, #120592, #73454, .T. ) ;
#10505=PLANE ( 'NONE',  #83096 ) ;
#10506=DIRECTION ( 'NONE',  ( 0.000000000000000000, 1.000000000000000000, 0.000000000000000000 ) ) ;
#10507=CARTESIAN_POINT ( 'NONE',  ( 9.599999999999917932, 12.50000000000000000, -2.276824562219559311E-15 ) ) ;
#10508=CARTESIAN_POINT ( 'NONE',  ( 6.249999999999934275, 12.50000000000000000, -7.122917578226816815 ) ) ;
#10509=DIRECTION ( 'NONE',  ( -4.274815082592931898E-19, -0.9999939076577903929, -0.003490651415223739937 ) ) ;
#10510=DIRECTION ( 'NONE',  ( -0.000000000000000000, 1.000000000000000000, -0.000000000000000000 ) ) ;
#10511=ADVANCED_FACE ( 'NONE', ( #870 ), #117336, .T. ) ;
#10512=EDGE_CURVE ( 'NONE', #38024, #5090, #44205, .T. ) ;
#10513=CARTESIAN_POINT ( 'NONE',  ( -1.050000000000037348, 12.50000000000000000, -2.511473670974877948 ) ) ;
#10514=VECTOR ( 'NONE', #43776, 1000.000000000000000 ) ;
#10515=ORIENTED_EDGE ( 'NONE', *, *, #107886, .F. ) ;
#10516=EDGE_CURVE ( 'NONE', #12146, #51476, #48328, .T. ) ;
#10517=CARTESIAN_POINT ( 'NONE',  ( 10.39999999999991509, 12.50000000000000000, 0.6277270498435120194 ) ) ;
#10518=EDGE_CURVE ( 'NONE', #123828, #126113, #72838, .T. ) ;
#10520=ORIENTED_EDGE ( 'NONE', *, *, #58411, .T. ) ;
#10521=ADVANCED_FACE ( 'NONE', ( #32293 ), #35953, .T. ) ;
#10522=DIRECTION ( 'NONE',  ( 0.000000000000000000, 0.000000000000000000, 1.000000000000000000 ) ) ;
#10523=CARTESIAN_POINT ( 'NONE',  ( -12.09999999999999609, 12.50000000000000000, 4.395220292106234439 ) ) ;
#10524=VECTOR ( 'NONE', #43921, 1000.000000000000000 ) ;
#10525=DIRECTION ( 'NONE',  ( -0.000000000000000000, 1.000000000000000000, -0.000000000000000000 ) ) ;
#10526=AXIS2_PLACEMENT_3D ( 'NONE', #68553, #88844, #109108 ) ;
#10527=DIRECTION ( 'NONE',  ( 0.000000000000000000, 0.000000000000000000, 1.000000000000000000 ) ) ;
#10528=DIRECTION ( 'NONE',  ( 0.000000000000000000, 0.000000000000000000, -1.000000000000000000 ) ) ;
#10529=DIRECTION ( 'NONE',  ( 0.000000000000000000, 1.000000000000000000, 0.000000000000000000 ) ) ;
#10530=ORIENTED_EDGE ( 'NONE', *, *, #38710, .T. ) ;
#10531=CONICAL_SURFACE ( 'NONE', #69024, 0.09999999999999999167, 0.003490658503988666988 ) ;
#10532=EDGE_LOOP ( 'NONE', ( #41848, #38167, #63814, #124519 ) ) ;
#10533=FACE_OUTER_BOUND ( 'NONE', #26316, .T. ) ;
#10534=VERTEX_POINT ( 'NONE', #70259 ) ;
#10535=DIRECTION ( 'NONE',  ( -0.000000000000000000, -1.000000000000000000, -0.000000000000000000 ) ) ;
#10536=CIRCLE ( 'NONE', #156, 0.1000000000000000472 ) ;
#10537=ORIENTED_EDGE ( 'NONE', *, *, #36366, .F. ) ;
#10539=CARTESIAN_POINT ( 'NONE',  ( 6.699999999999930012, 2.500000000000000000, 4.330127018922196314 ) ) ;
#10540=DIRECTION ( 'NONE',  ( -0.000000000000000000, -1.000000000000000000, -0.000000000000000000 ) ) ;
#10541=DIRECTION ( 'NONE',  ( 0.000000000000000000, 0.000000000000000000, -1.000000000000000000 ) ) ;
#10542=PLANE ( 'NONE',  #96680 ) ;
#10543=DIRECTION ( 'NONE',  ( 0.000000000000000000, 0.000000000000000000, -1.000000000000000000 ) ) ;
#10544=ORIENTED_EDGE ( 'NONE', *, *, #5060, .F. ) ;
#10545=CARTESIAN_POINT ( 'NONE',  ( 13.14999999999990088, 2.500000000000000000, 2.411473670974873862 ) ) ;
#10546=DIRECTION ( 'NONE',  ( 0.000000000000000000, 1.000000000000000000, 0.000000000000000000 ) ) ;
#10547=FACE_OUTER_BOUND ( 'NONE', #45300, .T. ) ;
#10548=CARTESIAN_POINT ( 'NONE',  ( -12.94999999999999218, 12.50000000000000000, 2.165063509461101265 ) ) ;
#10549=DIRECTION ( 'NONE',  ( 0.000000000000000000, 1.000000000000000000, 0.000000000000000000 ) ) ;
#10550=VERTEX_POINT ( 'NONE', #23089 ) ;
#10551=EDGE_LOOP ( 'NONE', ( #100498, #23386 ) ) ;
#10552=AXIS2_PLACEMENT_3D ( 'NONE', #67834, #18085, #58032 ) ;
#10554=DIRECTION ( 'NONE',  ( -0.000000000000000000, 1.000000000000000000, -0.000000000000000000 ) ) ;
#10555=ADVANCED_FACE ( 'NONE', ( #12605 ), #71535, .T. ) ;
#10556=AXIS2_PLACEMENT_3D ( 'NONE', #82337, #101966, #53517 ) ;
#10557=EDGE_CURVE ( 'NONE', #82548, #37370, #10050, .T. ) ;
#10558=EDGE_LOOP ( 'NONE', ( #44370, #73680 ) ) ;
#10559=DIRECTION ( 'NONE',  ( -4.274815082592931898E-19, -0.9999939076577903929, -0.003490651415223739937 ) ) ;
#10560=DIRECTION ( 'NONE',  ( 0.000000000000000000, 0.000000000000000000, -1.000000000000000000 ) ) ;
#10561=EDGE_CURVE ( 'NONE', #115875, #14684, #72202, .T. ) ;
#10562=ADVANCED_FACE ( 'NONE', ( #22466 ), #73594, .T. ) ;
#10563=VERTEX_POINT ( 'NONE', #61745 ) ;
#10564=CARTESIAN_POINT ( 'NONE',  ( 10.19999999999991225, 2.500000000000000000, -4.676537180435978769 ) ) ;
#10565=LINE ( 'NONE', #22358, #49568 ) ;
#10566=FACE_OUTER_BOUND ( 'NONE', #35032, .T. ) ;
#10567=CARTESIAN_POINT ( 'NONE',  ( -14.34999999999998543, 2.500000000000000000, -2.611473670974875372 ) ) ;
#10569=ADVANCED_FACE ( 'NONE', ( #51916 ), #125819, .T. ) ;
#10570=DIRECTION ( 'NONE',  ( 0.000000000000000000, 0.000000000000000000, 1.000000000000000000 ) ) ;
#10571=VERTEX_POINT ( 'NONE', #120642 ) ;
#10572=CARTESIAN_POINT ( 'NONE',  ( 48.83464596124490953, 3.619824809942020050, -4.313880784154338954 ) ) ;
#10573=DIRECTION ( 'NONE',  ( 0.000000000000000000, 0.000000000000000000, 1.000000000000000000 ) ) ;
#10574=EDGE_CURVE ( 'NONE', #90660, #15503, #31005, .T. ) ;
#10575=DIRECTION ( 'NONE',  ( 0.000000000000000000, -0.9999939076577903929, 0.003490651415223739937 ) ) ;
#10576=DIRECTION ( 'NONE',  ( 0.000000000000000000, 0.000000000000000000, -1.000000000000000000 ) ) ;
#10577=VERTEX_POINT ( 'NONE', #21146 ) ;
#10578=ORIENTED_EDGE ( 'NONE', *, *, #37774, .F. ) ;
#10579=LINE ( 'NONE', #80644, #79422 ) ;
#10580=CARTESIAN_POINT ( 'NONE',  ( -12.89999999999999147, 2.500000000000000000, 4.330127018922196314 ) ) ;
#10581=DIRECTION ( 'NONE',  ( 0.000000000000000000, 1.000000000000000000, 0.000000000000000000 ) ) ;
#10582=VERTEX_POINT ( 'NONE', #61076 ) ;
#10583=VECTOR ( 'NONE', #60940, 1000.000000000000000 ) ;
#10584=FACE_OUTER_BOUND ( 'NONE', #111600, .T. ) ;
#10585=AXIS2_PLACEMENT_3D ( 'NONE', #59504, #79752, #79125 ) ;
#10586=CARTESIAN_POINT ( 'NONE',  ( -7.100000000000017408, 12.50000000000000000, 0.6928203230275494784 ) ) ;
#10587=EDGE_LOOP ( 'NONE', ( #57060, #77842, #67948, #47811 ) ) ;
#10588=DIRECTION ( 'NONE',  ( 0.000000000000000000, 1.000000000000000000, 0.000000000000000000 ) ) ;
#10589=ORIENTED_EDGE ( 'NONE', *, *, #26245, .F. ) ;
#10590=CONICAL_SURFACE ( 'NONE', #31549, 0.09999999999999982514, 0.003490658503988666988 ) ;
#10591=CARTESIAN_POINT ( 'NONE',  ( 1.649999999999949729, 12.50000000000000000, 7.122917578226811486 ) ) ;
#10592=EDGE_LOOP ( 'NONE', ( #28315, #82445 ) ) ;
#10593=DIRECTION ( 'NONE',  ( 0.000000000000000000, 0.000000000000000000, -1.000000000000000000 ) ) ;
#10594=CARTESIAN_POINT ( 'NONE',  ( 15.40649769635636979, 2.500000000000000444, -5.817321165395405558 ) ) ;
#10595=EDGE_LOOP ( 'NONE', ( #82146, #93912, #35349, #126249 ) ) ;
#10596=VERTEX_POINT ( 'NONE', #11335 ) ;
#10597=CARTESIAN_POINT ( 'NONE',  ( 5.599999999999934808, 2.500000000000000000, -4.083716857408426826 ) ) ;
#10598=CARTESIAN_POINT ( 'NONE',  ( 5.199999999999935341, 2.500000000000000000, -3.983716857408426293 ) ) ;
#10599=ORIENTED_EDGE ( 'NONE', *, *, #116495, .F. ) ;
#10600=DIRECTION ( 'NONE',  ( 0.000000000000000000, 1.000000000000000000, 0.000000000000000000 ) ) ;
#10601=DIRECTION ( 'NONE',  ( 0.000000000000000000, 1.000000000000000000, 0.000000000000000000 ) ) ;
#10602=AXIS2_PLACEMENT_3D ( 'NONE', #65815, #94629, #14136 ) ;
#10604=CARTESIAN_POINT ( 'NONE',  ( 12.89999999999989910, 12.50000000000000000, 0.6277270498435120194 ) ) ;
#10605=CARTESIAN_POINT ( 'NONE',  ( 4.999999999999936939, 12.50000000000000000, -3.637306695894650055 ) ) ;
#10606=DIRECTION ( 'NONE',  ( 0.000000000000000000, 0.000000000000000000, 1.000000000000000000 ) ) ;
#10607=DIRECTION ( 'NONE',  ( 0.000000000000000000, 0.000000000000000000, 1.000000000000000000 ) ) ;
#10608=CARTESIAN_POINT ( 'NONE',  ( -4.150000000000025224, 2.500000000000000000, 7.188010851410848723 ) ) ;
#10609=VERTEX_POINT ( 'NONE', #74769 ) ;
#10610=ORIENTED_EDGE ( 'NONE', *, *, #14501, .T. ) ;
#10612=CONICAL_SURFACE ( 'NONE', #42042, 0.1000000000000000472, 0.003490658503988666988 ) ;
#10613=DIRECTION ( 'NONE',  ( -0.000000000000000000, 1.000000000000000000, -0.000000000000000000 ) ) ;
#10614=DIRECTION ( 'NONE',  ( -0.000000000000000000, -1.000000000000000000, -0.000000000000000000 ) ) ;
#10615=DIRECTION ( 'NONE',  ( 0.000000000000000000, 0.000000000000000000, -1.000000000000000000 ) ) ;
#10616=ORIENTED_EDGE ( 'NONE', *, *, #71564, .F. ) ;
#10617=ORIENTED_EDGE ( 'NONE', *, *, #24648, .T. ) ;
#10618=FACE_BOUND ( 'NONE', #33593, .T. ) ;
#10619=ORIENTED_EDGE ( 'NONE', *, *, #53836, .T. ) ;
#10620=DIRECTION ( 'NONE',  ( 0.000000000000000000, 0.000000000000000000, 1.000000000000000000 ) ) ;
#10621=DIRECTION ( 'NONE',  ( -0.000000000000000000, 1.000000000000000000, -0.000000000000000000 ) ) ;
#10622=CARTESIAN_POINT ( 'NONE',  ( -12.49999999999999467, 12.50000000000000000, -3.637306695894647390 ) ) ;
#10623=DIRECTION ( 'NONE',  ( 0.000000000000000000, -0.9999939076577903929, 0.003490651415223739937 ) ) ;
#10624=DIRECTION ( 'NONE',  ( -0.000000000000000000, -1.000000000000000000, -0.000000000000000000 ) ) ;
#10625=DIRECTION ( 'NONE',  ( 0.000000000000000000, 0.000000000000000000, -1.000000000000000000 ) ) ;
#10626=CARTESIAN_POINT ( 'NONE',  ( 8.149999999999923972, 12.50000000000000000, 1.818653347947321475 ) ) ;
#10627=DIRECTION ( 'NONE',  ( 0.000000000000000000, 0.000000000000000000, 1.000000000000000000 ) ) ;
#10628=DIRECTION ( 'NONE',  ( 0.000000000000000000, -0.000000000000000000, 1.000000000000000000 ) ) ;
#10629=LINE ( 'NONE', #80703, #15938 ) ;
#10630=ORIENTED_EDGE ( 'NONE', *, *, #59727, .T. ) ;
#10631=VERTEX_POINT ( 'NONE', #25020 ) ;
#10632=VERTEX_POINT ( 'NONE', #55761 ) ;
#10633=ORIENTED_EDGE ( 'NONE', *, *, #25517, .T. ) ;
#10634=FACE_OUTER_BOUND ( 'NONE', #126451, .T. ) ;
#10635=LINE ( 'NONE', #51896, #117616 ) ;
#10636=CIRCLE ( 'NONE', #121466, 0.06509327318403743123 ) ;
#10637=EDGE_LOOP ( 'NONE', ( #33843, #96447 ) ) ;
#10638=ORIENTED_EDGE ( 'NONE', *, *, #128169, .T. ) ;
#10640=LINE ( 'NONE', #49336, #37574 ) ;
#10641=EDGE_CURVE ( 'NONE', #1523, #54360, #115344, .T. ) ;
#10642=AXIS2_PLACEMENT_3D ( 'NONE', #43927, #83824, #13140 ) ;
#10643=FACE_OUTER_BOUND ( 'NONE', #14836, .T. ) ;
#10644=CARTESIAN_POINT ( 'NONE',  ( 0.000000000000000000, 0.000000000000000000, 0.000000000000000000 ) ) ;
#10645=CARTESIAN_POINT ( 'NONE',  ( -3.750000000000031086, 2.500000000000000000, -5.802370205355749988 ) ) ;
#10646=CARTESIAN_POINT ( 'NONE',  ( 3.149999999999946176, 2.500000000000000000, -6.741600689897077281 ) ) ;
#10647=CARTESIAN_POINT ( 'NONE',  ( 2.500000000000002220, 2.500000000000000000, 9.261799387799150907 ) ) ;
#10648=AXIS2_PLACEMENT_3D ( 'NONE', #99878, #18726, #8892 ) ;
#10649=CARTESIAN_POINT ( 'NONE',  ( 11.69999999999990870, 12.50000000000000000, 4.395220292106234439 ) ) ;
#10650=EDGE_CURVE ( 'NONE', #70505, #39225, #104890, .T. ) ;
#10651=VERTEX_POINT ( 'NONE', #36136 ) ;
#10652=ADVANCED_FACE ( 'NONE', ( #13245 ), #17130, .T. ) ;
#10653=CARTESIAN_POINT ( 'NONE',  ( -5.200000000000022382, 2.500000000000000000, 0.2464101615137735679 ) ) ;
#10654=VERTEX_POINT ( 'NONE', #105519 ) ;
#10655=ORIENTED_EDGE ( 'NONE', *, *, #53564, .F. ) ;
#10656=ORIENTED_EDGE ( 'NONE', *, *, #82969, .F. ) ;
#10657=EDGE_CURVE ( 'NONE', #122805, #39278, #38003, .T. ) ;
#10658=DIRECTION ( 'NONE',  ( 0.000000000000000000, 0.000000000000000000, -1.000000000000000000 ) ) ;
#10659=EDGE_CURVE ( 'NONE', #74338, #54151, #45318, .T. ) ;
#10660=EDGE_CURVE ( 'NONE', #108138, #24484, #26320, .T. ) ;
#10661=EDGE_LOOP ( 'NONE', ( #60121, #21797 ) ) ;
#10662=EDGE_CURVE ( 'NONE', #70366, #72904, #123756, .T. ) ;
#10663=EDGE_CURVE ( 'NONE', #114904, #35443, #75642, .T. ) ;
#10664=ORIENTED_EDGE ( 'NONE', *, *, #48165, .F. ) ;
#10667=CARTESIAN_POINT ( 'NONE',  ( -3.350000000000031619, 2.500000000000000000, -7.088010851410853519 ) ) ;
#10668=CARTESIAN_POINT ( 'NONE',  ( -10.80000000000000071, 12.50000000000000000, 0.06509327318403515528 ) ) ;
#10669=LINE ( 'NONE', #1511, #123611 ) ;
#10670=CARTESIAN_POINT ( 'NONE',  ( -4.999999999999990230, 12.50000000000000000, -4.330127018922201643 ) ) ;
#10671=DIRECTION ( 'NONE',  ( 0.000000000000000000, 1.000000000000000000, 0.000000000000000000 ) ) ;
#10672=ADVANCED_FACE ( 'NONE', ( #4704 ), #83924, .T. ) ;
#10673=CARTESIAN_POINT ( 'NONE',  ( 13.29999999999990301, 2.500000000000000000, 4.330127018922196314 ) ) ;
#10674=CIRCLE ( 'NONE', #14870, 0.06509327318403745899 ) ;
#10675=EDGE_CURVE ( 'NONE', #43290, #20224, #34863, .T. ) ;
#10676=AXIS2_PLACEMENT_3D ( 'NONE', #37110, #116927, #97310 ) ;
#10677=VERTEX_POINT ( 'NONE', #114678 ) ;
#10678=ORIENTED_EDGE ( 'NONE', *, *, #93773, .T. ) ;
#10679=CARTESIAN_POINT ( 'NONE',  ( 9.149999999999920419, 2.500000000000000000, 2.857883832488649301 ) ) ;
#10680=FACE_OUTER_BOUND ( 'NONE', #54665, .T. ) ;
#10681=ORIENTED_EDGE ( 'NONE', *, *, #124698, .F. ) ;
#10682=CARTESIAN_POINT ( 'NONE',  ( -3.350000000000031619, 2.500000000000000000, -5.702370205355749455 ) ) ;
#10683=CARTESIAN_POINT ( 'NONE',  ( -4.150000000000025224, 2.500000000000000000, 7.288010851410849256 ) ) ;
#10684=EDGE_LOOP ( 'NONE', ( #129611, #10396, #228, #107681 ) ) ;
#10685=CONICAL_SURFACE ( 'NONE', #4416, 0.09999999999999982514, 0.003490658503988666988 ) ;
#10686=CONICAL_SURFACE ( 'NONE', #108895, 0.09999999999999982514, 0.003490658503988666988 ) ;
#10687=DIRECTION ( 'NONE',  ( 0.000000000000000000, -0.9999939076577903929, 0.003490651415223739937 ) ) ;
#10688=EDGE_LOOP ( 'NONE', ( #47845, #110115 ) ) ;
#10689=ORIENTED_EDGE ( 'NONE', *, *, #5632, .F. ) ;
#10690=DIRECTION ( 'NONE',  ( -4.274815082592931898E-19, -0.9999939076577903929, -0.003490651415223739937 ) ) ;
#10691=DIRECTION ( 'NONE',  ( -0.000000000000000000, 1.000000000000000000, -0.000000000000000000 ) ) ;
#10692=CARTESIAN_POINT ( 'NONE',  ( -1.650000000000034772, 12.50000000000000000, 2.099970236277060032 ) ) ;
#10693=DIRECTION ( 'NONE',  ( 0.000000000000000000, -0.000000000000000000, 1.000000000000000000 ) ) ;
#10694=CONICAL_SURFACE ( 'NONE', #113118, 0.09999999999999982514, 0.003490658503988666988 ) ;
#10695=CIRCLE ( 'NONE', #25371, 0.1000000000000002554 ) ;
#10696=CARTESIAN_POINT ( 'NONE',  ( 5.649999999999934630, 2.500000000000000000, 6.148780366869520897 ) ) ;
#10698=CARTESIAN_POINT ( 'NONE',  ( -8.550000000000007816, 12.50000000000000000, 6.213873640053558134 ) ) ;
#10699=EDGE_CURVE ( 'NONE', #42755, #21163, #127892, .T. ) ;
#10700=ADVANCED_FACE ( 'NONE', ( #13896 ), #85225, .T. ) ;
#10701=VERTEX_POINT ( 'NONE', #55125 ) ;
#10702=CARTESIAN_POINT ( 'NONE',  ( -11.84999999999999609, 2.500000000000000000, 2.411473670974873862 ) ) ;
#10703=DIRECTION ( 'NONE',  ( 0.000000000000000000, 0.000000000000000000, 1.000000000000000000 ) ) ;
#10704=EDGE_CURVE ( 'NONE', #16035, #48618, #50616, .T. ) ;
#10705=AXIS2_PLACEMENT_3D ( 'NONE', #99019, #87884, #78093 ) ;
#10706=CIRCLE ( 'NONE', #4438, 0.09999999999999982514 ) ;
#10708=DIRECTION ( 'NONE',  ( 0.000000000000000000, -0.9999939076577903929, 0.003490651415223739937 ) ) ;
#10709=DIRECTION ( 'NONE',  ( -0.000000000000000000, -1.000000000000000000, -0.000000000000000000 ) ) ;
#10710=ADVANCED_FACE ( 'NONE', ( #115975 ), #53206, .T. ) ;
#10711=CARTESIAN_POINT ( 'NONE',  ( 10.84999999999990905, 2.500000000000000000, 1.372243186433545370 ) ) ;
#10713=EDGE_LOOP ( 'NONE', ( #53905, #115457 ) ) ;
#10714=ADVANCED_FACE ( 'NONE', ( #3444 ), #90306, .T. ) ;
#10715=DIRECTION ( 'NONE',  ( -0.000000000000000000, 1.000000000000000000, -0.000000000000000000 ) ) ;
#10716=EDGE_CURVE ( 'NONE', #74312, #27189, #29697, .T. ) ;
#10717=DIRECTION ( 'NONE',  ( -0.000000000000000000, -1.000000000000000000, -0.000000000000000000 ) ) ;
#10718=FACE_OUTER_BOUND ( 'NONE', #60015, .T. ) ;
#10719=EDGE_LOOP ( 'NONE', ( #55411, #61029, #45707, #39880 ) ) ;
#10720=EDGE_CURVE ( 'NONE', #56841, #123082, #117235, .T. ) ;
#10721=DIRECTION ( 'NONE',  ( -0.000000000000000000, 1.000000000000000000, -0.000000000000000000 ) ) ;
#10722=ORIENTED_EDGE ( 'NONE', *, *, #36268, .F. ) ;
#10723=ORIENTED_EDGE ( 'NONE', *, *, #82134, .F. ) ;
#10724=DIRECTION ( 'NONE',  ( 0.000000000000000000, 0.000000000000000000, 1.000000000000000000 ) ) ;
#10725=AXIS2_PLACEMENT_3D ( 'NONE', #27427, #105362, #88948 ) ;
#10726=AXIS2_PLACEMENT_3D ( 'NONE', #65082, #54002, #14689 ) ;
#10727=VERTEX_POINT ( 'NONE', #67493 ) ;
#10729=FACE_OUTER_BOUND ( 'NONE', #107087, .T. ) ;
#10730=EDGE_LOOP ( 'NONE', ( #88628, #25723 ) ) ;
#10731=AXIS2_PLACEMENT_3D ( 'NONE', #94956, #65472, #77867 ) ;
#10732=CARTESIAN_POINT ( 'NONE',  ( -6.650000000000018119, 12.50000000000000000, -7.188010851410854052 ) ) ;
#10733=CIRCLE ( 'NONE', #25410, 0.1000000000000002554 ) ;
#10734=FACE_OUTER_BOUND ( 'NONE', #116078, .T. ) ;
#10735=VECTOR ( 'NONE', #35020, 1000.000000000000000 ) ;
#10736=DIRECTION ( 'NONE',  ( 0.000000000000000000, 1.000000000000000000, 0.000000000000000000 ) ) ;
#10737=ADVANCED_FACE ( 'NONE', ( #47896 ), #119557, .T. ) ;
#10738=EDGE_LOOP ( 'NONE', ( #9690, #40134, #37091, #123826 ) ) ;
#10739=EDGE_LOOP ( 'NONE', ( #68036, #16677, #76196, #53537 ) ) ;
#10740=VERTEX_POINT ( 'NONE', #76699 ) ;
#10741=FACE_OUTER_BOUND ( 'NONE', #54431, .T. ) ;
#10742=FACE_OUTER_BOUND ( 'NONE', #119104, .T. ) ;
#10743=DIRECTION ( 'NONE',  ( 0.000000000000000000, 1.000000000000000000, 0.000000000000000000 ) ) ;
#10744=FACE_BOUND ( 'NONE', #127212, .T. ) ;
#10745=ORIENTED_EDGE ( 'NONE', *, *, #58487, .F. ) ;
#10746=LINE ( 'NONE', #121369, #67894 ) ;
#10747=CARTESIAN_POINT ( 'NONE',  ( -1.050000000000038680, 12.50000000000000000, 2.511473670974873507 ) ) ;
#10748=ORIENTED_EDGE ( 'NONE', *, *, #84745, .F. ) ;
#10749=DIRECTION ( 'NONE',  ( 0.000000000000000000, -0.9999939076577903929, 0.003490651415223739937 ) ) ;
#10750=LINE ( 'NONE', #30450, #67976 ) ;
#10751=ADVANCED_FACE ( 'NONE', ( #108079 ), #16468, .T. ) ;
#10752=CARTESIAN_POINT ( 'NONE',  ( 12.29999999999990301, 2.500000000000000000, -0.3464101615137782364 ) ) ;
#10753=DIRECTION ( 'NONE',  ( 0.000000000000000000, 1.000000000000000000, 0.000000000000000000 ) ) ;
#10754=DIRECTION ( 'NONE',  ( 0.000000000000000000, 1.000000000000000000, 0.000000000000000000 ) ) ;
#10755=CARTESIAN_POINT ( 'NONE',  ( 11.89999999999990798, 12.50000000000000000, -4.611443907251939756 ) ) ;
#10756=CARTESIAN_POINT ( 'NONE',  ( -14.14999999999998614, 2.500000000000000000, 2.165063509461101265 ) ) ;
#10758=AXIS2_PLACEMENT_3D ( 'NONE', #68332, #30366, #120663 ) ;
#10759=VERTEX_POINT ( 'NONE', #66222 ) ;
#10760=VERTEX_POINT ( 'NONE', #38067 ) ;
#10761=EDGE_LOOP ( 'NONE', ( #6609, #14538 ) ) ;
#10762=VERTEX_POINT ( 'NONE', #39380 ) ;
#10763=CARTESIAN_POINT ( 'NONE',  ( 11.89999999999990443, 2.500000000000000000, -0.3464101615137782364 ) ) ;
#10765=EDGE_LOOP ( 'NONE', ( #127914, #49127, #24922, #34068 ) ) ;
#10766=EDGE_CURVE ( 'NONE', #26528, #3892, #23422, .T. ) ;
#10767=FACE_BOUND ( 'NONE', #21816, .T. ) ;
#10768=CONICAL_SURFACE ( 'NONE', #127873, 0.09999999999999982514, 0.003490658503988666988 ) ;
#10769=CARTESIAN_POINT ( 'NONE',  ( 6.249999999999932498, 2.500000000000000000, 5.702370205355745014 ) ) ;
#10770=CONICAL_SURFACE ( 'NONE', #4504, 0.09999999999999982514, 0.003490658503988666988 ) ;
#10771=CARTESIAN_POINT ( 'NONE',  ( 14.99999999999989342, 2.500000000000000000, -0.6928203230275541413 ) ) ;
#10772=AXIS2_PLACEMENT_3D ( 'NONE', #48236, #117589, #105870 ) ;
#10773=PLANE ( 'NONE',  #3158 ) ;
#10774=DIRECTION ( 'NONE',  ( 0.000000000000000000, 0.000000000000000000, -1.000000000000000000 ) ) ;
#10775=CARTESIAN_POINT ( 'NONE',  ( 14.79999999999989235, 12.50000000000000000, 0.3464101615137735735 ) ) ;
#10777=DIRECTION ( 'NONE',  ( -4.274815082592931898E-19, -0.9999939076577903929, -0.003490651415223739937 ) ) ;
#10778=FACE_OUTER_BOUND ( 'NONE', #80822, .T. ) ;
#10779=DIRECTION ( 'NONE',  ( 0.000000000000000000, 0.000000000000000000, 1.000000000000000000 ) ) ;
#10780=ORIENTED_EDGE ( 'NONE', *, *, #96681, .T. ) ;
#10781=VECTOR ( 'NONE', #93342, 1000.000000000000000 ) ;
#10782=ORIENTED_EDGE ( 'NONE', *, *, #123892, .F. ) ;
#10783=CIRCLE ( 'NONE', #44252, 0.06509327318403745899 ) ;
#10784=VERTEX_POINT ( 'NONE', #126454 ) ;
#10785=ORIENTED_EDGE ( 'NONE', *, *, #77814, .F. ) ;
#10786=ORIENTED_EDGE ( 'NONE', *, *, #10990, .F. ) ;
#10787=ORIENTED_EDGE ( 'NONE', *, *, #90608, .T. ) ;
#10788=CIRCLE ( 'NONE', #119468, 0.06509327318403745899 ) ;
#10789=CARTESIAN_POINT ( 'NONE',  ( 6.249999999999932498, 12.50000000000000000, -2.792790559304616504 ) ) ;
#10790=EDGE_LOOP ( 'NONE', ( #104052, #13089, #11313, #6444 ) ) ;
#10791=EDGE_CURVE ( 'NONE', #74876, #2020, #27613, .T. ) ;
#10792=CARTESIAN_POINT ( 'NONE',  ( -10.85000000000000142, 2.500000000000000000, 6.595190528383296780 ) ) ;
#10793=CONICAL_SURFACE ( 'NONE', #119567, 0.09999999999999999167, 0.003490658503988666988 ) ;
#10794=VECTOR ( 'NONE', #109037, 1000.000000000000000 ) ;
#10796=FACE_OUTER_BOUND ( 'NONE', #96872, .T. ) ;
#10797=DIRECTION ( 'NONE',  ( -0.000000000000000000, -1.000000000000000000, -0.000000000000000000 ) ) ;
#10798=VERTEX_POINT ( 'NONE', #97625 ) ;
#10799=CARTESIAN_POINT ( 'NONE',  ( -12.69999999999999218, 2.500000000000000000, -4.576537180435974683 ) ) ;
#10800=EDGE_CURVE ( 'NONE', #97332, #64242, #44355, .T. ) ;
#10801=VERTEX_POINT ( 'NONE', #66865 ) ;
#10802=EDGE_LOOP ( 'NONE', ( #77142, #125439, #22246, #44843 ) ) ;
#10803=FACE_OUTER_BOUND ( 'NONE', #27578, .T. ) ;
#10804=ADVANCED_FACE ( 'NONE', ( #79291 ), #77792, .T. ) ;
#10805=DIRECTION ( 'NONE',  ( -4.274815082592931898E-19, -0.9999939076577903929, -0.003490651415223739937 ) ) ;
#10806=DIRECTION ( 'NONE',  ( -4.274815082592931898E-19, -0.9999939076577903929, -0.003490651415223739937 ) ) ;
#10807=EDGE_CURVE ( 'NONE', #13428, #20160, #4612, .T. ) ;
#10808=ADVANCED_FACE ( 'NONE', ( #98258 ), #71435, .T. ) ;
#10809=EDGE_CURVE ( 'NONE', #79461, #98821, #94430, .T. ) ;
#10810=ORIENTED_EDGE ( 'NONE', *, *, #98310, .T. ) ;
#10811=ORIENTED_EDGE ( 'NONE', *, *, #65834, .T. ) ;
#10813=CARTESIAN_POINT ( 'NONE',  ( 5.449999999999937117, 12.50000000000000000, -6.495190528383302464 ) ) ;
#10814=EDGE_CURVE ( 'NONE', #63398, #69417, #31842, .T. ) ;
#10815=DIRECTION ( 'NONE',  ( 0.000000000000000000, -0.9999939076577903929, 0.003490651415223739937 ) ) ;
#10816=AXIS2_PLACEMENT_3D ( 'NONE', #1908, #10445, #111879 ) ;
#10817=CARTESIAN_POINT ( 'NONE',  ( -9.800000000000006040, 2.500000000000000000, 0.3464101615137735735 ) ) ;
#10818=ORIENTED_EDGE ( 'NONE', *, *, #44863, .T. ) ;
#10819=AXIS2_PLACEMENT_3D ( 'NONE', #128754, #78997, #90734 ) ;
#10820=AXIS2_PLACEMENT_3D ( 'NONE', #55136, #23751, #95065 ) ;
#10821=B_SPLINE_CURVE_WITH_KNOTS ( 'NONE', 3,
 ( #98586, #61274, #49524, #110359, #89434, #100534, #101194, #71083 ),
 .UNSPECIFIED., .F., .F.,
 ( 4, 2, 2, 4 ),
 ( 0.002994103107820098031, 0.003957537843903998452, 0.004920972579987898873, 0.006847842052155699716 ),
 .UNSPECIFIED. ) ;
#10822=LINE ( 'NONE', #20681, #4200 ) ;
#10823=EDGE_CURVE ( 'NONE', #28983, #34057, #127723, .T. ) ;
#10824=ORIENTED_EDGE ( 'NONE', *, *, #85053, .T. ) ;
#10825=LINE ( 'NONE', #100515, #25987 ) ;
#10826=ADVANCED_FACE ( 'NONE', ( #68156 ), #121712, .T. ) ;
#10827=AXIS2_PLACEMENT_3D ( 'NONE', #54230, #11716, #121667 ) ;
#10829=ORIENTED_EDGE ( 'NONE', *, *, #125053, .F. ) ;
#10830=CARTESIAN_POINT ( 'NONE',  ( 17.50000000000000000, 2.500000000000000000, 4.000000000000000000 ) ) ;
#10831=CIRCLE ( 'NONE', #98667, 0.06509327318403745899 ) ;
#10832=CARTESIAN_POINT ( 'NONE',  ( 81.97074409615474622, -3.937872622146114221, 6.123955080831738229 ) ) ;
#10833=CARTESIAN_POINT ( 'NONE',  ( -10.40000000000000213, 2.500000000000000000, 0.7928203230275495672 ) ) ;
#10834=CIRCLE ( 'NONE', #42266, 0.06509327318403745899 ) ;
#10835=DIRECTION ( 'NONE',  ( -0.000000000000000000, 1.000000000000000000, -0.000000000000000000 ) ) ;
#10836=EDGE_CURVE ( 'NONE', #26300, #67411, #119658, .T. ) ;
#10837=ORIENTED_EDGE ( 'NONE', *, *, #33947, .F. ) ;
#10838=CIRCLE ( 'NONE', #84008, 0.09999999999999982514 ) ;
#10839=DIRECTION ( 'NONE',  ( 0.000000000000000000, -0.9999939076577903929, 0.003490651415223739937 ) ) ;
#10840=CARTESIAN_POINT ( 'NONE',  ( -2.700000000000029932, 12.50000000000000000, -4.741630453620015118 ) ) ;
#10841=ORIENTED_EDGE ( 'NONE', *, *, #55764, .F. ) ;
#10842=ORIENTED_EDGE ( 'NONE', *, *, #114460, .T. ) ;
#10843=ORIENTED_EDGE ( 'NONE', *, *, #122751, .T. ) ;
#10844=CARTESIAN_POINT ( 'NONE',  ( 10.59999999999990905, 12.50000000000000000, 4.676537180435972552 ) ) ;
#10846=CARTESIAN_POINT ( 'NONE',  ( 2.499999999999945377, 2.500000000000000000, 4.922947341949748257 ) ) ;
#10847=DIRECTION ( 'NONE',  ( 0.000000000000000000, 1.000000000000000000, 0.000000000000000000 ) ) ;
#10848=DIRECTION ( 'NONE',  ( -0.000000000000000000, 1.000000000000000000, -0.000000000000000000 ) ) ;
#10849=DIRECTION ( 'NONE',  ( -0.000000000000000000, -1.000000000000000000, -0.000000000000000000 ) ) ;
#10850=DIRECTION ( 'NONE',  ( -0.000000000000000000, 1.000000000000000000, -0.000000000000000000 ) ) ;
#10851=DIRECTION ( 'NONE',  ( -0.000000000000000000, -1.000000000000000000, -0.000000000000000000 ) ) ;
#10852=LINE ( 'NONE', #8291, #38040 ) ;
#10853=AXIS2_PLACEMENT_3D ( 'NONE', #34422, #123413, #92676 ) ;
#10854=CIRCLE ( 'NONE', #21343, 0.06509327318403745899 ) ;
#10855=ORIENTED_EDGE ( 'NONE', *, *, #76135, .F. ) ;
#10856=CARTESIAN_POINT ( 'NONE',  ( -8.950000000000004619, 2.500000000000000000, 6.048780366869521252 ) ) ;
#10857=DIRECTION ( 'NONE',  ( 0.000000000000000000, 0.000000000000000000, -1.000000000000000000 ) ) ;
#10858=DIRECTION ( 'NONE',  ( 0.000000000000000000, 1.000000000000000000, 0.000000000000000000 ) ) ;
#10859=FACE_OUTER_BOUND ( 'NONE', #119418, .T. ) ;
#10860=AXIS2_PLACEMENT_3D ( 'NONE', #126834, #19443, #47630 ) ;
#10861=AXIS2_PLACEMENT_3D ( 'NONE', #50144, #71059, #12756 ) ;
#10862=ORIENTED_EDGE ( 'NONE', *, *, #54967, .F. ) ;
#10863=DIRECTION ( 'NONE',  ( 0.000000000000000000, 1.000000000000000000, 0.000000000000000000 ) ) ;
#10864=ADVANCED_FACE ( 'NONE', ( #58996 ), #71546, .T. ) ;
#10865=AXIS2_PLACEMENT_3D ( 'NONE', #54495, #94414, #114703 ) ;
#10866=AXIS2_PLACEMENT_3D ( 'NONE', #17294, #47442, #106978 ) ;
#10867=EDGE_CURVE ( 'NONE', #70927, #30745, #13030, .T. ) ;
#10868=DIRECTION ( 'NONE',  ( -0.000000000000000000, 1.000000000000000000, -0.000000000000000000 ) ) ;
#10869=DIRECTION ( 'NONE',  ( 0.000000000000000000, 1.000000000000000000, 0.000000000000000000 ) ) ;
#10870=EDGE_LOOP ( 'NONE', ( #38015, #121632 ) ) ;
#10871=CIRCLE ( 'NONE', #111227, 0.06509327318403745899 ) ;
#10872=ORIENTED_EDGE ( 'NONE', *, *, #61935, .F. ) ;
#10873=EDGE_CURVE ( 'NONE', #102784, #15089, #62225, .T. ) ;
#10874=DIRECTION ( 'NONE',  ( 0.000000000000000000, 0.000000000000000000, 1.000000000000000000 ) ) ;
#10875=AXIS2_PLACEMENT_3D ( 'NONE', #61001, #21076, #29610 ) ;
#10876=EDGE_LOOP ( 'NONE', ( #14427, #11680, #110711, #127759 ) ) ;
#10877=AXIS2_PLACEMENT_3D ( 'NONE', #10598, #88531, #99006 ) ;
#10878=AXIS2_PLACEMENT_3D ( 'NONE', #93763, #64293, #7946 ) ;
#10880=AXIS2_PLACEMENT_3D ( 'NONE', #124487, #125743, #104816 ) ;
#10881=DIRECTION ( 'NONE',  ( -0.000000000000000000, -1.000000000000000000, -0.000000000000000000 ) ) ;
#10882=CIRCLE ( 'NONE', #59040, 0.09999999999999982514 ) ;
#10883=DIRECTION ( 'NONE',  ( 0.000000000000000000, 1.000000000000000000, 0.000000000000000000 ) ) ;
#10884=DIRECTION ( 'NONE',  ( 0.000000000000000000, 1.000000000000000000, 0.000000000000000000 ) ) ;
#10885=CARTESIAN_POINT ( 'NONE',  ( -6.050000000000018474, 12.50000000000000000, 6.776507416713035248 ) ) ;
#10886=VERTEX_POINT ( 'NONE', #20992 ) ;
#10887=CONICAL_SURFACE ( 'NONE', #23434, 0.1000000000000002554, 0.003490658503988666988 ) ;
#10888=FACE_OUTER_BOUND ( 'NONE', #104389, .T. ) ;
#10889=VERTEX_POINT ( 'NONE', #40664 ) ;
#10890=CARTESIAN_POINT ( 'NONE',  ( 16.73289298692834492, 0.7002450284443078043, 5.897165230072824116 ) ) ;
#10891=DIRECTION ( 'NONE',  ( 0.000000000000000000, 1.000000000000000000, 0.000000000000000000 ) ) ;
#10892=EDGE_LOOP ( 'NONE', ( #24681, #83998, #116537, #71270 ) ) ;
#10893=ORIENTED_EDGE ( 'NONE', *, *, #33180, .T. ) ;
#10894=EDGE_LOOP ( 'NONE', ( #62682, #127832 ) ) ;
#10895=ORIENTED_EDGE ( 'NONE', *, *, #107631, .T. ) ;
#10896=CARTESIAN_POINT ( 'NONE',  ( 0.3999999999999563904, 2.500000000000000000, 3.637306695894644726 ) ) ;
#10897=DIRECTION ( 'NONE',  ( 0.000000000000000000, 0.000000000000000000, -1.000000000000000000 ) ) ;
#10898=DIRECTION ( 'NONE',  ( 0.000000000000000000, 0.000000000000000000, 1.000000000000000000 ) ) ;
#10899=FACE_BOUND ( 'NONE', #16600, .T. ) ;
#10900=CARTESIAN_POINT ( 'NONE',  ( 4.599999999999937472, 2.500000000000000000, 0.7928203230275495672 ) ) ;
#10902=DIRECTION ( 'NONE',  ( 0.000000000000000000, 0.000000000000000000, -1.000000000000000000 ) ) ;
#10903=CARTESIAN_POINT ( 'NONE',  ( -5.650000000000019895, 2.500000000000000000, 2.511473670974873507 ) ) ;
#10904=CONICAL_SURFACE ( 'NONE', #69418, 0.1000000000000000472, 0.003490658503988666988 ) ;
#10905=AXIS2_PLACEMENT_3D ( 'NONE', #78045, #125217, #116674 ) ;
#10906=CARTESIAN_POINT ( 'NONE',  ( -12.94999999999999218, 12.50000000000000000, -2.165063509461099489 ) ) ;
#10907=AXIS2_PLACEMENT_3D ( 'NONE', #1356, #20368, #69448 ) ;
#10908=DIRECTION ( 'NONE',  ( 0.000000000000000000, -0.000000000000000000, 1.000000000000000000 ) ) ;
#10909=CARTESIAN_POINT ( 'NONE',  ( 11.89999999999990798, 2.500000000000000000, -3.883716857408426648 ) ) ;
#10910=CONICAL_SURFACE ( 'NONE', #17168, 0.1000000000000002554, 0.003490658503988666988 ) ;
#10911=AXIS2_PLACEMENT_3D ( 'NONE', #117115, #125021, #26185 ) ;
#10912=FACE_OUTER_BOUND ( 'NONE', #58568, .T. ) ;
#10913=VECTOR ( 'NONE', #38048, 1000.000000000000000 ) ;
#10914=ORIENTED_EDGE ( 'NONE', *, *, #20478, .T. ) ;
#10915=EDGE_LOOP ( 'NONE', ( #106284, #71012, #54914, #88635 ) ) ;
#10916=ORIENTED_EDGE ( 'NONE', *, *, #66892, .T. ) ;
#10917=ORIENTED_EDGE ( 'NONE', *, *, #23704, .F. ) ;
#10918=VECTOR ( 'NONE', #6768, 1000.000000000000000 ) ;
#10919=EDGE_CURVE ( 'NONE', #61864, #44929, #69481, .T. ) ;
#10920=DIRECTION ( 'NONE',  ( 0.000000000000000000, 0.000000000000000000, 1.000000000000000000 ) ) ;
#10921=CIRCLE ( 'NONE', #52808, 0.1000000000000002554 ) ;
#10922=CARTESIAN_POINT ( 'NONE',  ( 105.5000000000000142, -1.500000000000000222, -1.322875655532295136 ) ) ;
#10923=ORIENTED_EDGE ( 'NONE', *, *, #87822, .F. ) ;
#10924=ADVANCED_FACE ( 'NONE', ( #90365 ), #29781, .T. ) ;
#10925=FACE_BOUND ( 'NONE', #13229, .T. ) ;
#10926=AXIS2_PLACEMENT_3D ( 'NONE', #22808, #62726, #20853 ) ;
#10927=DIRECTION ( 'NONE',  ( 0.000000000000000000, -0.000000000000000000, 1.000000000000000000 ) ) ;
#10928=ORIENTED_EDGE ( 'NONE', *, *, #125660, .T. ) ;
#10929=CARTESIAN_POINT ( 'NONE',  ( -9.150000000000009237, 12.50000000000000000, 1.537336459617582918 ) ) ;
#10930=CARTESIAN_POINT ( 'NONE',  ( -6.250000000000021316, 2.500000000000000000, -5.702370205355749455 ) ) ;
#10931=ADVANCED_FACE ( 'NONE', ( #60917 ), #89738, .T. ) ;
#10932=DIRECTION ( 'NONE',  ( 0.000000000000000000, 0.000000000000000000, 1.000000000000000000 ) ) ;
#10933=FACE_OUTER_BOUND ( 'NONE', #2957, .T. ) ;
#10934=EDGE_LOOP ( 'NONE', ( #25257, #54587, #106461, #27104 ) ) ;
#10935=DIRECTION ( 'NONE',  ( -0.000000000000000000, 1.000000000000000000, -0.000000000000000000 ) ) ;
#10936=AXIS2_PLACEMENT_3D ( 'NONE', #48764, #97205, #48112 ) ;
#10937=ORIENTED_EDGE ( 'NONE', *, *, #77809, .F. ) ;
#10938=EDGE_LOOP ( 'NONE', ( #7864, #29800 ) ) ;
#10939=CARTESIAN_POINT ( 'NONE',  ( 8.099999999999923261, 12.50000000000000000, -3.983716857408426293 ) ) ;
#10940=CARTESIAN_POINT ( 'NONE',  ( -5.800000000000018474, 2.500000000000000000, 4.430127018922196847 ) ) ;
#10941=VERTEX_POINT ( 'NONE', #10517 ) ;
#10942=DIRECTION ( 'NONE',  ( 0.000000000000000000, 0.000000000000000000, 1.000000000000000000 ) ) ;
#10943=CIRCLE ( 'NONE', #36120, 0.06509327318403745899 ) ;
#10944=STYLED_ITEM ( 'NONE', ( #84767 ), #58374 ) ;
#10945=DIRECTION ( 'NONE',  ( 0.000000000000000000, 0.000000000000000000, 1.000000000000000000 ) ) ;
#10946=DIRECTION ( 'NONE',  ( -0.000000000000000000, 1.000000000000000000, -0.000000000000000000 ) ) ;
#10947=ADVANCED_FACE ( 'NONE', ( #9890 ), #92477, .T. ) ;
#10948=CARTESIAN_POINT ( 'NONE',  ( 12.29999999999990656, 2.500000000000000000, 3.983716857408420964 ) ) ;
#10949=ORIENTED_EDGE ( 'NONE', *, *, #67403, .T. ) ;
#10950=CARTESIAN_POINT ( 'NONE',  ( -11.64999999999999680, 2.500000000000000000, -2.857883832488649745 ) ) ;
#10951=AXIS2_PLACEMENT_3D ( 'NONE', #39613, #59245, #57945 ) ;
#10952=ORIENTED_EDGE ( 'NONE', *, *, #48216, .F. ) ;
#10953=DIRECTION ( 'NONE',  ( 0.000000000000000000, 0.000000000000000000, 1.000000000000000000 ) ) ;
#10954=CONICAL_SURFACE ( 'NONE', #115414, 0.1000000000000000472, 0.003490658503988666988 ) ;
#10955=AXIS2_PLACEMENT_3D ( 'NONE', #108841, #11290, #110146 ) ;
#10956=ADVANCED_FACE ( 'NONE', ( #82511 ), #102141, .T. ) ;
#10958=AXIS2_PLACEMENT_3D ( 'NONE', #36352, #7499, #78197 ) ;
#10959=PLANE ( 'NONE',  #93544 ) ;
#10961=DIRECTION ( 'NONE',  ( 0.000000000000000000, 0.000000000000000000, 1.000000000000000000 ) ) ;
#10962=CARTESIAN_POINT ( 'NONE',  ( 8.149999999999920419, 12.50000000000000000, -2.511473670974877948 ) ) ;
#10963=EDGE_CURVE ( 'NONE', #65382, #113506, #49833, .T. ) ;
#10964=CARTESIAN_POINT ( 'NONE',  ( 8.349999999999919709, 12.50000000000000000, 7.188010851410848723 ) ) ;
#10965=DIRECTION ( 'NONE',  ( 0.000000000000000000, -0.000000000000000000, 1.000000000000000000 ) ) ;
#10966=EDGE_CURVE ( 'NONE', #53057, #107141, #61178, .T. ) ;
#10967=EDGE_CURVE ( 'NONE', #34976, #52139, #96662, .T. ) ;
#10968=DIRECTION ( 'NONE',  ( 0.000000000000000000, 0.000000000000000000, 1.000000000000000000 ) ) ;
#10969=ADVANCED_FACE ( 'NONE', ( #19714 ), #11166, .T. ) ;
#10970=AXIS2_PLACEMENT_3D ( 'NONE', #48434, #98172, #30755 ) ;
#10971=ORIENTED_EDGE ( 'NONE', *, *, #487, .F. ) ;
#10972=EDGE_LOOP ( 'NONE', ( #89741, #81144, #33266, #127752 ) ) ;
#10973=AXIS2_PLACEMENT_3D ( 'NONE', #39320, #79223, #39941 ) ;
#10974=EDGE_LOOP ( 'NONE', ( #75182, #26315, #90798, #73399 ) ) ;
#10975=LINE ( 'NONE', #120947, #76934 ) ;
#10976=FACE_OUTER_BOUND ( 'NONE', #68668, .T. ) ;
#10978=CONICAL_SURFACE ( 'NONE', #115436, 0.1000000000000002554, 0.003490658503988666988 ) ;
#10979=CIRCLE ( 'NONE', #48666, 0.1000000000000002554 ) ;
#10980=EDGE_CURVE ( 'NONE', #27825, #50205, #51120, .T. ) ;
#10981=FACE_OUTER_BOUND ( 'NONE', #6371, .T. ) ;
#10982=ORIENTED_EDGE ( 'NONE', *, *, #7307, .F. ) ;
#10983=VERTEX_POINT ( 'NONE', #111286 ) ;
#10984=EDGE_LOOP ( 'NONE', ( #66985, #118411, #88207, #40553 ) ) ;
#10985=ADVANCED_FACE ( 'NONE', ( #30192 ), #75744, .T. ) ;
#10986=CARTESIAN_POINT ( 'NONE',  ( -6.850000000000017408, 12.50000000000000000, -6.841600689897077814 ) ) ;
#10987=AXIS2_PLACEMENT_3D ( 'NONE', #3860, #103365, #24155 ) ;
#10988=ORIENTED_EDGE ( 'NONE', *, *, #19548, .F. ) ;
#10989=DIRECTION ( 'NONE',  ( -0.000000000000000000, 1.000000000000000000, -0.000000000000000000 ) ) ;
#10990=EDGE_CURVE ( 'NONE', #48757, #97573, #94608, .T. ) ;
#10991=EDGE_CURVE ( 'NONE', #77648, #102955, #20358, .T. ) ;
#10992=DIRECTION ( 'NONE',  ( -0.000000000000000000, 1.000000000000000000, -0.000000000000000000 ) ) ;
#10993=AXIS2_PLACEMENT_3D ( 'NONE', #108674, #19660, #59611 ) ;
#10994=DIRECTION ( 'NONE',  ( -0.000000000000000000, 1.000000000000000000, -0.000000000000000000 ) ) ;
#10995=CARTESIAN_POINT ( 'NONE',  ( 1.649999999999951505, 12.50000000000000000, 1.537336459617582918 ) ) ;
#10996=CARTESIAN_POINT ( 'NONE',  ( -9.150000000000009237, 2.500000000000000000, -2.265063509461101798 ) ) ;
#10997=DIRECTION ( 'NONE',  ( 0.000000000000000000, 0.000000000000000000, -1.000000000000000000 ) ) ;
#10999=DIRECTION ( 'NONE',  ( -0.000000000000000000, -1.000000000000000000, -0.000000000000000000 ) ) ;
#11000=ADVANCED_FACE ( 'NONE', ( #705 ), #522, .T. ) ;
#11001=ORIENTED_EDGE ( 'NONE', *, *, #48554, .T. ) ;
#11002=ORIENTED_EDGE ( 'NONE', *, *, #40574, .T. ) ;
#11003=CARTESIAN_POINT ( 'NONE',  ( -10.80000000000000071, 2.500000000000000000, -0.1000000000000022815 ) ) ;
#11005=VERTEX_POINT ( 'NONE', #54960 ) ;
#11006=ORIENTED_EDGE ( 'NONE', *, *, #56895, .F. ) ;
#11007=CIRCLE ( 'NONE', #126024, 0.09999999999999982514 ) ;
#11009=CARTESIAN_POINT ( 'NONE',  ( 1.899999999999949507, 2.500000000000000000, 4.676537180435972552 ) ) ;
#11010=DIRECTION ( 'NONE',  ( 0.000000000000000000, -0.9999939076577903929, 0.003490651415223739937 ) ) ;
#11011=CARTESIAN_POINT ( 'NONE',  ( -14.14999999999998792, 2.500000000000000000, -1.372243186433547812 ) ) ;
#11012=DIRECTION ( 'NONE',  ( -0.000000000000000000, 1.000000000000000000, -0.000000000000000000 ) ) ;
#11013=DIRECTION ( 'NONE',  ( 0.000000000000000000, 0.000000000000000000, -1.000000000000000000 ) ) ;
#11014=VECTOR ( 'NONE', #93857, 1000.000000000000000 ) ;
#11015=DIRECTION ( 'NONE',  ( -0.000000000000000000, -1.000000000000000000, -0.000000000000000000 ) ) ;
#11016=CARTESIAN_POINT ( 'NONE',  ( -1.900000000000034106, 2.500000000000000000, 0.2464101615137735679 ) ) ;
#11017=AXIS2_PLACEMENT_3D ( 'NONE', #102109, #51726, #122401 ) ;
#11018=AXIS2_PLACEMENT_3D ( 'NONE', #30534, #96177, #20696 ) ;
#11019=FACE_OUTER_BOUND ( 'NONE', #128007, .T. ) ;
#11020=EDGE_LOOP ( 'NONE', ( #59276, #58185, #81162, #50206 ) ) ;
#11021=AXIS2_PLACEMENT_3D ( 'NONE', #110037, #60309, #100212 ) ;
#11022=EDGE_LOOP ( 'NONE', ( #32612, #54673, #14738, #102572 ) ) ;
#11023=AXIS2_PLACEMENT_3D ( 'NONE', #128601, #109581, #68997 ) ;
#11024=ORIENTED_EDGE ( 'NONE', *, *, #96532, .T. ) ;
#11025=AXIS2_PLACEMENT_3D ( 'NONE', #56215, #57526, #43372 ) ;
#11026=AXIS2_PLACEMENT_3D ( 'NONE', #92138, #111796, #102601 ) ;
#11027=AXIS2_PLACEMENT_3D ( 'NONE', #95358, #89240, #19865 ) ;
#11028=EDGE_LOOP ( 'NONE', ( #97553, #124010 ) ) ;
#11029=ORIENTED_EDGE ( 'NONE', *, *, #83308, .F. ) ;
#11030=FACE_OUTER_BOUND ( 'NONE', #55435, .T. ) ;
#11031=DIRECTION ( 'NONE',  ( 0.000000000000000000, 1.000000000000000000, 0.000000000000000000 ) ) ;
#11032=VECTOR ( 'NONE', #71087, 1000.000000000000000 ) ;
#11033=EDGE_LOOP ( 'NONE', ( #79626, #43338, #121142, #37243 ) ) ;
#11034=DIRECTION ( 'NONE',  ( 0.000000000000000000, -0.9999939076577903929, 0.003490651415223739937 ) ) ;
#11035=EDGE_CURVE ( 'NONE', #85157, #29857, #98722, .T. ) ;
#11036=FACE_OUTER_BOUND ( 'NONE', #98318, .T. ) ;
#11037=EDGE_CURVE ( 'NONE', #117332, #48425, #64778, .T. ) ;
#11038=DIRECTION ( 'NONE',  ( 0.000000000000000000, 1.000000000000000000, 0.000000000000000000 ) ) ;
#11039=CARTESIAN_POINT ( 'NONE',  ( -9.600000000000008527, 12.50000000000000000, -4.330127018922197202 ) ) ;
#11040=VERTEX_POINT ( 'NONE', #85070 ) ;
#11041=DIRECTION ( 'NONE',  ( 0.000000000000000000, 0.000000000000000000, 1.000000000000000000 ) ) ;
#11042=DIRECTION ( 'NONE',  ( 0.000000000000000000, 1.000000000000000000, 0.000000000000000000 ) ) ;
#11043=ORIENTED_EDGE ( 'NONE', *, *, #7436, .F. ) ;
#11044=ORIENTED_EDGE ( 'NONE', *, *, #116070, .F. ) ;
#11045=ORIENTED_EDGE ( 'NONE', *, *, #20915, .F. ) ;
#11046=VERTEX_POINT ( 'NONE', #62855 ) ;
#11047=DIRECTION ( 'NONE',  ( 0.000000000000000000, 0.000000000000000000, 1.000000000000000000 ) ) ;
#11048=CARTESIAN_POINT ( 'NONE',  ( -9.150000000000009237, 2.500000000000000000, -7.088010851410848190 ) ) ;
#11049=AXIS2_PLACEMENT_3D ( 'NONE', #106213, #16517, #97031 ) ;
#11050=DIRECTION ( 'NONE',  ( 0.000000000000000000, -0.9999939076577903929, 0.003490651415223739937 ) ) ;
#11051=CIRCLE ( 'NONE', #23584, 0.09999999999999982514 ) ;
#11052=DIRECTION ( 'NONE',  ( 0.000000000000000000, 0.000000000000000000, 1.000000000000000000 ) ) ;
#11053=VERTEX_POINT ( 'NONE', #13088 ) ;
#11054=CARTESIAN_POINT ( 'NONE',  ( 9.149999999999916866, 12.50000000000000000, 7.122917578226811486 ) ) ;
#11055=CARTESIAN_POINT ( 'NONE',  ( 20.80940928220344688, -0.7000174339600981899, -4.161255421338320382 ) ) ;
#11056=LINE ( 'NONE', #39910, #278 ) ;
#11057=DIRECTION ( 'NONE',  ( 0.000000000000000000, 0.000000000000000000, 1.000000000000000000 ) ) ;
#11058=CIRCLE ( 'NONE', #15248, 0.1000000000000000472 ) ;
#11059=AXIS2_PLACEMENT_3D ( 'NONE', #88942, #39227, #37901 ) ;
#11060=AXIS2_PLACEMENT_3D ( 'NONE', #47860, #7909, #25614 ) ;
#11061=EDGE_LOOP ( 'NONE', ( #14258, #29682, #87909, #93982 ) ) ;
#11062=AXIS2_PLACEMENT_3D ( 'NONE', #66272, #6676, #46634 ) ;
#11063=EDGE_LOOP ( 'NONE', ( #53079, #15574 ) ) ;
#11064=ORIENTED_EDGE ( 'NONE', *, *, #110064, .F. ) ;
#11065=DIRECTION ( 'NONE',  ( 0.000000000000000000, 0.000000000000000000, 1.000000000000000000 ) ) ;
#11066=CARTESIAN_POINT ( 'NONE',  ( -1.650000000000035660, 2.500000000000000000, 2.957883832488649389 ) ) ;
#11067=FACE_BOUND ( 'NONE', #72849, .T. ) ;
#11068=CARTESIAN_POINT ( 'NONE',  ( -13.34999999999999076, 12.50000000000000000, 2.857883832488652853 ) ) ;
#11069=AXIS2_PLACEMENT_3D ( 'NONE', #3217, #21557, #43158 ) ;
#11070=DIRECTION ( 'NONE',  ( 0.000000000000000000, -0.000000000000000000, 1.000000000000000000 ) ) ;
#11071=CIRCLE ( 'NONE', #111131, 0.1000000000000002554 ) ;
#11072=CARTESIAN_POINT ( 'NONE',  ( -15.19999999999998330, 12.50000000000000000, 0.3464101615137758494 ) ) ;
#11073=EDGE_CURVE ( 'NONE', #66202, #128693, #38202, .T. ) ;
#11074=CIRCLE ( 'NONE', #617, 0.06509327318403745899 ) ;
#11075=CONICAL_SURFACE ( 'NONE', #82206, 0.1000000000000002554, 0.003490658503988666988 ) ;
#11076=CARTESIAN_POINT ( 'NONE',  ( 0.7999999999999553024, 12.50000000000000000, -4.330127018922201643 ) ) ;
#11077=DIRECTION ( 'NONE',  ( -4.274815082592931898E-19, -0.9999939076577903929, -0.003490651415223739937 ) ) ;
#11078=AXIS2_PLACEMENT_3D ( 'NONE', #28671, #9665, #68576 ) ;
#11080=ORIENTED_EDGE ( 'NONE', *, *, #23802, .T. ) ;
#11081=DIRECTION ( 'NONE',  ( 0.000000000000000000, 1.000000000000000000, 0.000000000000000000 ) ) ;
#11082=CARTESIAN_POINT ( 'NONE',  ( 2.299999999999947864, 12.50000000000000000, 3.918623584224383727 ) ) ;
#11083=AXIS2_PLACEMENT_3D ( 'NONE', #18849, #19497, #109153 ) ;
#11084=ORIENTED_EDGE ( 'NONE', *, *, #105579, .T. ) ;
#11085=ORIENTED_EDGE ( 'NONE', *, *, #43784, .F. ) ;
#11086=ADVANCED_FACE ( 'NONE', ( #45161 ), #53681, .T. ) ;
#11087=FACE_OUTER_BOUND ( 'NONE', #58184, .T. ) ;
#11088=CARTESIAN_POINT ( 'NONE',  ( 15.79999999999989058, 12.50000000000000000, -2.385244779468109755E-15 ) ) ;
#11089=EDGE_CURVE ( 'NONE', #4826, #44047, #65275, .T. ) ;
#11090=FACE_BOUND ( 'NONE', #56302, .T. ) ;
#11091=CARTESIAN_POINT ( 'NONE',  ( 15.62915144542246004, -2.500000000000000444, -5.624002559040088833 ) ) ;
#11092=FACE_OUTER_BOUND ( 'NONE', #28171, .T. ) ;
#11093=CONICAL_SURFACE ( 'NONE', #48687, 0.09999999999999982514, 0.003490658503988666988 ) ;
#11094=ORIENTED_EDGE ( 'NONE', *, *, #77282, .T. ) ;
#11095=DIRECTION ( 'NONE',  ( 0.000000000000000000, -0.9999939076577903929, 0.003490651415223739937 ) ) ;
#11096=AXIS2_PLACEMENT_3D ( 'NONE', #119708, #1229, #40539 ) ;
#11097=EDGE_CURVE ( 'NONE', #126294, #114390, #111322, .T. ) ;
#11098=DIRECTION ( 'NONE',  ( -4.274815082592931898E-19, -0.9999939076577903929, -0.003490651415223739937 ) ) ;
#11099=ORIENTED_EDGE ( 'NONE', *, *, #13287, .T. ) ;
#11100=CARTESIAN_POINT ( 'NONE',  ( -4.150000000000024336, 2.500000000000000000, 1.472243186433545459 ) ) ;
#11101=DIRECTION ( 'NONE',  ( 0.000000000000000000, 1.000000000000000000, 0.000000000000000000 ) ) ;
#11102=AXIS2_PLACEMENT_3D ( 'NONE', #4277, #74983, #75608 ) ;
#11103=VECTOR ( 'NONE', #11095, 1000.000000000000000 ) ;
#11104=AXIS2_PLACEMENT_3D ( 'NONE', #92784, #22128, #3114 ) ;
#11105=AXIS2_PLACEMENT_3D ( 'NONE', #78834, #97163, #99754 ) ;
#11106=DIRECTION ( 'NONE',  ( 0.000000000000000000, 0.000000000000000000, -1.000000000000000000 ) ) ;
#11107=CARTESIAN_POINT ( 'NONE',  ( -9.150000000000005684, 2.500000000000000000, 7.188010851410848723 ) ) ;
#11108=CONICAL_SURFACE ( 'NONE', #44583, 0.09999999999999982514, 0.003490658503988666988 ) ;
#11109=AXIS2_PLACEMENT_3D ( 'NONE', #67872, #19410, #8304 ) ;
#11110=EDGE_LOOP ( 'NONE', ( #12604, #50491, #24644, #25817 ) ) ;
#11111=CIRCLE ( 'NONE', #17367, 0.1000000000000002554 ) ;
#11112=FACE_OUTER_BOUND ( 'NONE', #128764, .T. ) ;
#11113=FACE_OUTER_BOUND ( 'NONE', #85102, .T. ) ;
#11114=CARTESIAN_POINT ( 'NONE',  ( 2.899999999999945732, 2.500000000000000000, 0.09999999999999761857 ) ) ;
#11115=VECTOR ( 'NONE', #101318, 1000.000000000000000 ) ;
#11116=ORIENTED_EDGE ( 'NONE', *, *, #99395, .F. ) ;
#11117=ORIENTED_EDGE ( 'NONE', *, *, #64113, .F. ) ;
#11118=DIRECTION ( 'NONE',  ( -0.000000000000000000, -1.000000000000000000, -0.000000000000000000 ) ) ;
#11119=AXIS2_PLACEMENT_3D ( 'NONE', #40693, #11189, #98942 ) ;
#11121=DIRECTION ( 'NONE',  ( 0.000000000000000000, -0.9999939076577903929, 0.003490651415223739937 ) ) ;
#11122=CARTESIAN_POINT ( 'NONE',  ( 3.749999999999978684, 2.500000000000000000, -6.495190528383302464 ) ) ;
#11123=EDGE_CURVE ( 'NONE', #844, #126108, #3927, .T. ) ;
#11124=DIRECTION ( 'NONE',  ( -4.274815082592931898E-19, -0.9999939076577903929, -0.003490651415223739937 ) ) ;
#11125=ORIENTED_EDGE ( 'NONE', *, *, #127782, .T. ) ;
#11126=DIRECTION ( 'NONE',  ( -0.000000000000000000, -1.000000000000000000, -0.000000000000000000 ) ) ;
#11127=CARTESIAN_POINT ( 'NONE',  ( -7.950000000000012612, 2.500000000000000000, 2.165063509461097713 ) ) ;
#11128=DIRECTION ( 'NONE',  ( -4.274815082592931898E-19, -0.9999939076577903929, -0.003490651415223739937 ) ) ;
#11129=DIRECTION ( 'NONE',  ( 0.000000000000000000, 0.000000000000000000, 1.000000000000000000 ) ) ;
#11130=PLANE ( 'NONE',  #77884 ) ;
#11131=ADVANCED_FACE ( 'NONE', ( #35337 ), #10978, .T. ) ;
#11132=CARTESIAN_POINT ( 'NONE',  ( 3.149999999999946176, 2.500000000000000000, -6.841600689897077814 ) ) ;
#11133=EDGE_CURVE ( 'NONE', #46899, #33469, #113229, .T. ) ;
#11134=VECTOR ( 'NONE', #65654, 1000.000000000000000 ) ;
#11136=ORIENTED_EDGE ( 'NONE', *, *, #52627, .T. ) ;
#11138=EDGE_LOOP ( 'NONE', ( #49901, #1675 ) ) ;
#11139=DIRECTION ( 'NONE',  ( 0.000000000000000000, 0.000000000000000000, 1.000000000000000000 ) ) ;
#11140=EDGE_CURVE ( 'NONE', #8844, #120440, #19301, .T. ) ;
#11141=ORIENTED_EDGE ( 'NONE', *, *, #18972, .F. ) ;
#11142=EDGE_LOOP ( 'NONE', ( #87301, #41231, #105542, #3784 ) ) ;
#11143=ADVANCED_FACE ( 'NONE', ( #73965 ), #84424, .T. ) ;
#11144=EDGE_LOOP ( 'NONE', ( #23408, #72454, #100022, #39450 ) ) ;
#11145=EDGE_CURVE ( 'NONE', #12263, #47265, #23571, .T. ) ;
#11146=DIRECTION ( 'NONE',  ( 0.000000000000000000, 0.000000000000000000, -1.000000000000000000 ) ) ;
#11147=ADVANCED_FACE ( 'NONE', ( #103428 ), #73779, .T. ) ;
#11148=VECTOR ( 'NONE', #4432, 1000.000000000000000 ) ;
#11149=CIRCLE ( 'NONE', #40427, 0.06509327318403741736 ) ;
#11150=LINE ( 'NONE', #29520, #125860 ) ;
#11151=AXIS2_PLACEMENT_3D ( 'NONE', #16404, #55713, #95644 ) ;
#11152=DIRECTION ( 'NONE',  ( -0.000000000000000000, 1.000000000000000000, -0.000000000000000000 ) ) ;
#11154=ADVANCED_FACE ( 'NONE', ( #5848 ), #34087, .T. ) ;
#11155=DIRECTION ( 'NONE',  ( 0.000000000000000000, -0.000000000000000000, 1.000000000000000000 ) ) ;
#11156=PLANE ( 'NONE',  #22953 ) ;
#11157=CARTESIAN_POINT ( 'NONE',  ( 9.349999999999916156, 12.50000000000000000, 6.148780366869520009 ) ) ;
#11158=CARTESIAN_POINT ( 'NONE',  ( -6.900000000000015454, 2.500000000000000000, 4.676537180435972552 ) ) ;
#11159=FACE_OUTER_BOUND ( 'NONE', #24777, .T. ) ;
#11160=AXIS2_PLACEMENT_3D ( 'NONE', #24713, #104556, #14853 ) ;
#11161=CARTESIAN_POINT ( 'NONE',  ( -6.250000000000021316, 12.50000000000000000, -1.407149913249512663 ) ) ;
#11162=ADVANCED_FACE ( 'NONE', ( #122430 ), #2663, .T. ) ;
#11163=CIRCLE ( 'NONE', #98998, 0.06509327318403745899 ) ;
#11164=ORIENTED_EDGE ( 'NONE', *, *, #100403, .F. ) ;
#11165=AXIS2_PLACEMENT_3D ( 'NONE', #48912, #35379, #114563 ) ;
#11166=PLANE ( 'NONE',  #84141 ) ;
#11167=ORIENTED_EDGE ( 'NONE', *, *, #64785, .T. ) ;
#11168=VERTEX_POINT ( 'NONE', #72683 ) ;
#11169=DIRECTION ( 'NONE',  ( -0.000000000000000000, 1.000000000000000000, -0.000000000000000000 ) ) ;
#11170=CIRCLE ( 'NONE', #34466, 0.06509327318403745899 ) ;
#11171=DIRECTION ( 'NONE',  ( 0.000000000000000000, -0.9999939076577903929, 0.003490651415223739937 ) ) ;
#11172=CARTESIAN_POINT ( 'NONE',  ( -2.700000000000031264, 2.500000000000000000, 4.676537180435972552 ) ) ;
#11173=DIRECTION ( 'NONE',  ( 0.000000000000000000, 0.000000000000000000, 1.000000000000000000 ) ) ;
#11174=AXIS2_PLACEMENT_3D ( 'NONE', #101730, #41538, #4141 ) ;
#11176=AXIS2_PLACEMENT_3D ( 'NONE', #124691, #65752, #116784 ) ;
#11177=AXIS2_PLACEMENT_3D ( 'NONE', #24685, #63312, #103246 ) ;
#11178=DIRECTION ( 'NONE',  ( 0.000000000000000000, 1.000000000000000000, 0.000000000000000000 ) ) ;
#11179=VERTEX_POINT ( 'NONE', #94243 ) ;
#11180=AXIS2_PLACEMENT_3D ( 'NONE', #1611, #21923, #2924 ) ;
#11181=ORIENTED_EDGE ( 'NONE', *, *, #35411, .F. ) ;
#11182=CARTESIAN_POINT ( 'NONE',  ( 7.299999999999926104, 12.50000000000000000, -0.3464101615137782364 ) ) ;
#11183=ORIENTED_EDGE ( 'NONE', *, *, #115411, .F. ) ;
#11184=CARTESIAN_POINT ( 'NONE',  ( -14.14999999999998614, 2.500000000000000000, 1.472243186433549456 ) ) ;
#11185=EDGE_LOOP ( 'NONE', ( #13242, #101655, #80265, #129482 ) ) ;
#11186=VERTEX_POINT ( 'NONE', #124359 ) ;
#11187=FACE_OUTER_BOUND ( 'NONE', #83128, .T. ) ;
#11188=DIRECTION ( 'NONE',  ( -0.000000000000000000, 1.000000000000000000, -0.000000000000000000 ) ) ;
#11189=DIRECTION ( 'NONE',  ( -0.000000000000000000, -1.000000000000000000, -0.000000000000000000 ) ) ;
#11190=EDGE_CURVE ( 'NONE', #21419, #85535, #74609, .T. ) ;
#11191=FACE_OUTER_BOUND ( 'NONE', #14004, .T. ) ;
#11192=PLANE ( 'NONE',  #105695 ) ;
#11193=ORIENTED_EDGE ( 'NONE', *, *, #55792, .F. ) ;
#11194=CARTESIAN_POINT ( 'NONE',  ( -6.700000000000019718, 12.50000000000000000, -4.395220292106239768 ) ) ;
#11195=DIRECTION ( 'NONE',  ( 0.000000000000000000, 0.000000000000000000, 1.000000000000000000 ) ) ;
#11196=CIRCLE ( 'NONE', #86405, 0.06509327318403745899 ) ;
#11197=VECTOR ( 'NONE', #59541, 1000.000000000000000 ) ;
#11198=CARTESIAN_POINT ( 'NONE',  ( 14.79999999999989413, 2.500000000000000000, -0.3464101615137782364 ) ) ;
#11199=CARTESIAN_POINT ( 'NONE',  ( -13.54999999999998828, 2.500000000000000000, -2.411473670974875638 ) ) ;
#11200=PLANE ( 'NONE',  #14329 ) ;
#11201=EDGE_CURVE ( 'NONE', #30841, #91689, #42408, .T. ) ;
#11202=EDGE_LOOP ( 'NONE', ( #124036, #68654 ) ) ;
#11203=AXIS2_PLACEMENT_3D ( 'NONE', #99788, #121346, #270 ) ;
#11204=AXIS2_PLACEMENT_3D ( 'NONE', #60319, #19738, #59680 ) ;
#11205=VECTOR ( 'NONE', #100613, 1000.000000000000000 ) ;
#11206=ORIENTED_EDGE ( 'NONE', *, *, #108351, .F. ) ;
#11207=AXIS2_PLACEMENT_3D ( 'NONE', #128037, #78309, #48186 ) ;
#11209=CARTESIAN_POINT ( 'NONE',  ( -14.14999999999998792, 12.50000000000000000, 2.857883832488652853 ) ) ;
#11210=ORIENTED_EDGE ( 'NONE', *, *, #704, .T. ) ;
#11211=CARTESIAN_POINT ( 'NONE',  ( 17.49101023696819368, -2.144674160806593566, 4.220798295113220355 ) ) ;
#11212=DIRECTION ( 'NONE',  ( -0.000000000000000000, -1.000000000000000000, -0.000000000000000000 ) ) ;
#11213=AXIS2_PLACEMENT_3D ( 'NONE', #111326, #22346, #122475 ) ;
#11214=AXIS2_PLACEMENT_3D ( 'NONE', #112961, #1069, #23283 ) ;
#11215=AXIS2_PLACEMENT_3D ( 'NONE', #44103, #84020, #123946 ) ;
#11216=AXIS2_PLACEMENT_3D ( 'NONE', #56883, #117741, #77200 ) ;
#11217=ORIENTED_EDGE ( 'NONE', *, *, #37332, .F. ) ;
#11218=DIRECTION ( 'NONE',  ( 0.000000000000000000, 1.000000000000000000, 0.000000000000000000 ) ) ;
#11219=DIRECTION ( 'NONE',  ( 0.000000000000000000, 0.000000000000000000, -1.000000000000000000 ) ) ;
#11220=CARTESIAN_POINT ( 'NONE',  ( 12.29999999999990123, 2.500000000000000000, 0.2464101615137735679 ) ) ;
#11221=DIRECTION ( 'NONE',  ( 0.000000000000000000, 1.000000000000000000, 0.000000000000000000 ) ) ;
#11222=VERTEX_POINT ( 'NONE', #96169 ) ;
#11223=VERTEX_POINT ( 'NONE', #86999 ) ;
#11224=FACE_OUTER_BOUND ( 'NONE', #117702, .T. ) ;
#11225=LINE ( 'NONE', #51181, #35191 ) ;
#11226=DIRECTION ( 'NONE',  ( 0.000000000000000000, 1.000000000000000000, 0.000000000000000000 ) ) ;
#11227=DIRECTION ( 'NONE',  ( 0.000000000000000000, 0.000000000000000000, 1.000000000000000000 ) ) ;
#11228=ADVANCED_FACE ( 'NONE', ( #68003 ), #76545, .T. ) ;
#11229=ORIENTED_EDGE ( 'NONE', *, *, #76511, .T. ) ;
#11230=VERTEX_POINT ( 'NONE', #107285 ) ;
#11231=DIRECTION ( 'NONE',  ( -0.000000000000000000, 1.000000000000000000, -0.000000000000000000 ) ) ;
#11232=CARTESIAN_POINT ( 'NONE',  ( -8.350000000000013856, 12.50000000000000000, -2.230156782645139391 ) ) ;
#11233=LINE ( 'NONE', #1420, #83177 ) ;
#11234=AXIS2_PLACEMENT_3D ( 'NONE', #42982, #103156, #33143 ) ;
#11236=AXIS2_PLACEMENT_3D ( 'NONE', #89193, #127201, #97719 ) ;
#11237=EDGE_CURVE ( 'NONE', #740, #128936, #61281, .T. ) ;
#11238=AXIS2_PLACEMENT_3D ( 'NONE', #77561, #121197, #31538 ) ;
#11239=DIRECTION ( 'NONE',  ( 0.000000000000000000, 1.000000000000000000, 0.000000000000000000 ) ) ;
#11240=DIRECTION ( 'NONE',  ( 0.000000000000000000, 1.000000000000000000, 0.000000000000000000 ) ) ;
#11241=VERTEX_POINT ( 'NONE', #97469 ) ;
#11242=ADVANCED_FACE ( 'NONE', ( #46425 ), #126940, .T. ) ;
#11243=CARTESIAN_POINT ( 'NONE',  ( 11.84999999999990727, 2.500000000000000000, 6.941600689897073018 ) ) ;
#11244=VECTOR ( 'NONE', #51522, 1000.000000000000000 ) ;
#11247=LINE ( 'NONE', #120571, #83028 ) ;
#11248=VECTOR ( 'NONE', #93265, 1000.000000000000000 ) ;
#11249=ORIENTED_EDGE ( 'NONE', *, *, #101917, .T. ) ;
#11250=AXIS2_PLACEMENT_3D ( 'NONE', #106368, #118770, #16037 ) ;
#11251=ORIENTED_EDGE ( 'NONE', *, *, #14084, .T. ) ;
#11252=CARTESIAN_POINT ( 'NONE',  ( 12.89999999999989910, 12.50000000000000000, 0.6928203230275494784 ) ) ;
#11253=DIRECTION ( 'NONE',  ( 0.000000000000000000, 0.000000000000000000, -1.000000000000000000 ) ) ;
#11254=ADVANCED_FACE ( 'NONE', ( #17608 ), #77186, .T. ) ;
#11255=ORIENTED_EDGE ( 'NONE', *, *, #57398, .T. ) ;
#11256=ORIENTED_EDGE ( 'NONE', *, *, #6340, .T. ) ;
#11257=ADVANCED_FACE ( 'NONE', ( #67327 ), #75830, .T. ) ;
#11258=AXIS2_PLACEMENT_3D ( 'NONE', #39027, #88058, #38365 ) ;
#11259=CARTESIAN_POINT ( 'NONE',  ( -6.850000000000013856, 2.500000000000000000, 6.148780366869520897 ) ) ;
#11260=CARTESIAN_POINT ( 'NONE',  ( -9.800000000000006040, 12.50000000000000000, 0.2813168883297361700 ) ) ;
#11261=EDGE_LOOP ( 'NONE', ( #84158, #81235, #83157, #38821 ) ) ;
#11262=CARTESIAN_POINT ( 'NONE',  ( -0.2000000000000339284, 12.50000000000000000, -0.2813168883297385570 ) ) ;
#11264=VECTOR ( 'NONE', #57786, 1000.000000000000000 ) ;
#11265=CARTESIAN_POINT ( 'NONE',  ( 0.3999999999999563904, 12.50000000000000000, 5.022947341949748790 ) ) ;
#11266=VECTOR ( 'NONE', #29483, 1000.000000000000000 ) ;
#11267=AXIS2_PLACEMENT_3D ( 'NONE', #31147, #81521, #90689 ) ;
#11268=LINE ( 'NONE', #21089, #103664 ) ;
#11269=CARTESIAN_POINT ( 'NONE',  ( 1.449999999999952660, 12.50000000000000000, -6.841600689897078702 ) ) ;
#11270=CARTESIAN_POINT ( 'NONE',  ( -8.550000000000009592, 2.500000000000000000, 6.741600689897071952 ) ) ;
#11271=CONICAL_SURFACE ( 'NONE', #809, 0.09999999999999982514, 0.003490658503988666988 ) ;
#11272=CARTESIAN_POINT ( 'NONE',  ( -9.800000000000007816, 2.500000000000000000, -3.883716857408422207 ) ) ;
#11273=AXIS2_PLACEMENT_3D ( 'NONE', #57145, #29614, #48620 ) ;
#11274=ORIENTED_EDGE ( 'NONE', *, *, #64235, .F. ) ;
#11275=ORIENTED_EDGE ( 'NONE', *, *, #103759, .T. ) ;
#11276=DIRECTION ( 'NONE',  ( 0.000000000000000000, 1.000000000000000000, 0.000000000000000000 ) ) ;
#11277=ORIENTED_EDGE ( 'NONE', *, *, #118917, .F. ) ;
#11278=CARTESIAN_POINT ( 'NONE',  ( 6.649999999999930189, 2.500000000000000000, 5.702370205355745014 ) ) ;
#11279=DIRECTION ( 'NONE',  ( 0.000000000000000000, 0.000000000000000000, -1.000000000000000000 ) ) ;
#11280=DIRECTION ( 'NONE',  ( 0.000000000000000000, 0.000000000000000000, -1.000000000000000000 ) ) ;
#11282=ORIENTED_EDGE ( 'NONE', *, *, #121633, .T. ) ;
#11283=FACE_BOUND ( 'NONE', #118572, .T. ) ;
#11284=ORIENTED_EDGE ( 'NONE', *, *, #92391, .F. ) ;
#11285=DIRECTION ( 'NONE',  ( 0.000000000000000000, 0.000000000000000000, -1.000000000000000000 ) ) ;
#11286=CARTESIAN_POINT ( 'NONE',  ( 14.19999999999989626, 2.500000000000000000, -2.276824562219559311E-15 ) ) ;
#11287=DIRECTION ( 'NONE',  ( 0.000000000000000000, 1.000000000000000000, 0.000000000000000000 ) ) ;
#11288=DIRECTION ( 'NONE',  ( 0.000000000000000000, 0.000000000000000000, 1.000000000000000000 ) ) ;
#11289=CARTESIAN_POINT ( 'NONE',  ( 6.649999999999930189, 2.500000000000000000, -2.757883832488654097 ) ) ;
#11290=DIRECTION ( 'NONE',  ( -0.000000000000000000, 1.000000000000000000, -0.000000000000000000 ) ) ;
#11291=CIRCLE ( 'NONE', #59643, 0.06509327318403745899 ) ;
#11292=FACE_OUTER_BOUND ( 'NONE', #10043, .T. ) ;
#11293=CARTESIAN_POINT ( 'NONE',  ( 10.39999999999991509, 12.50000000000000000, -0.6928203230275542523 ) ) ;
#11294=AXIS2_PLACEMENT_3D ( 'NONE', #5690, #56710, #46266 ) ;
#11295=CIRCLE ( 'NONE', #7071, 0.09999999999999982514 ) ;
#11296=DIRECTION ( 'NONE',  ( -0.000000000000000000, 1.000000000000000000, -0.000000000000000000 ) ) ;
#11297=LINE ( 'NONE', #91157, #77793 ) ;
#11298=DIRECTION ( 'NONE',  ( -0.000000000000000000, 1.000000000000000000, -0.000000000000000000 ) ) ;
#11299=ADVANCED_FACE ( 'NONE', ( #56873 ), #113489, .T. ) ;
#11300=AXIS2_PLACEMENT_3D ( 'NONE', #25084, #33623, #53906 ) ;
#11301=CIRCLE ( 'NONE', #84470, 0.06509327318403745899 ) ;
#11302=ORIENTED_EDGE ( 'NONE', *, *, #10504, .F. ) ;
#11303=VERTEX_POINT ( 'NONE', #56249 ) ;
#11304=VERTEX_POINT ( 'NONE', #86345 ) ;
#11305=ORIENTED_EDGE ( 'NONE', *, *, #67516, .F. ) ;
#11306=DIRECTION ( 'NONE',  ( 0.000000000000000000, 0.000000000000000000, 1.000000000000000000 ) ) ;
#11307=CIRCLE ( 'NONE', #103256, 0.06509327318403745899 ) ;
#11309=LINE ( 'NONE', #79426, #54953 ) ;
#11310=EDGE_CURVE ( 'NONE', #121502, #107629, #63321, .T. ) ;
#11311=VERTEX_POINT ( 'NONE', #37902 ) ;
#11312=EDGE_LOOP ( 'NONE', ( #83722, #109539, #125198, #20072 ) ) ;
#11313=ORIENTED_EDGE ( 'NONE', *, *, #20040, .T. ) ;
#11314=EDGE_CURVE ( 'NONE', #6379, #101677, #8429, .T. ) ;
#11315=CARTESIAN_POINT ( 'NONE',  ( -8.300000000000011369, 2.500000000000000000, 0.09999999999999772959 ) ) ;
#11316=EDGE_CURVE ( 'NONE', #45963, #14446, #92566, .T. ) ;
#11317=AXIS2_PLACEMENT_3D ( 'NONE', #5733, #26045, #33925 ) ;
#11318=AXIS2_PLACEMENT_3D ( 'NONE', #9186, #49779, #89040 ) ;
#11319=DIRECTION ( 'NONE',  ( -0.000000000000000000, -1.000000000000000000, -0.000000000000000000 ) ) ;
#11320=DIRECTION ( 'NONE',  ( 0.000000000000000000, 1.000000000000000000, 0.000000000000000000 ) ) ;
#11321=FACE_OUTER_BOUND ( 'NONE', #56669, .T. ) ;
#11322=EDGE_CURVE ( 'NONE', #85535, #116043, #80053, .T. ) ;
#11323=CARTESIAN_POINT ( 'NONE',  ( 9.399999999999915090, 12.50000000000000000, -4.676537180435977881 ) ) ;
#11324=CARTESIAN_POINT ( 'NONE',  ( 13.09999999999990195, 12.50000000000000000, 3.983716857408420076 ) ) ;
#11325=CONICAL_SURFACE ( 'NONE', #15512, 0.09999999999999982514, 0.003490658503988666988 ) ;
#11326=DIRECTION ( 'NONE',  ( -0.000000000000000000, -1.000000000000000000, -0.000000000000000000 ) ) ;
#11327=ORIENTED_EDGE ( 'NONE', *, *, #28612, .T. ) ;
#11328=DIRECTION ( 'NONE',  ( 0.000000000000000000, 0.000000000000000000, 1.000000000000000000 ) ) ;
#11329=EDGE_CURVE ( 'NONE', #119031, #47664, #38577, .T. ) ;
#11330=EDGE_LOOP ( 'NONE', ( #42515, #105357, #107392, #75808 ) ) ;
#11331=EDGE_CURVE ( 'NONE', #27897, #24765, #84240, .T. ) ;
#11332=VERTEX_POINT ( 'NONE', #35973 ) ;
#11333=ORIENTED_EDGE ( 'NONE', *, *, #46921, .F. ) ;
#11334=AXIS2_PLACEMENT_3D ( 'NONE', #43383, #11326, #121926 ) ;
#11335=CARTESIAN_POINT ( 'NONE',  ( -3.749999999999991562, 2.500000000000000000, 6.395190528383296602 ) ) ;
#11336=ORIENTED_EDGE ( 'NONE', *, *, #37041, .T. ) ;
#11337=ORIENTED_EDGE ( 'NONE', *, *, #69954, .F. ) ;
#11338=ORIENTED_EDGE ( 'NONE', *, *, #82769, .F. ) ;
#11339=AXIS2_PLACEMENT_3D ( 'NONE', #37973, #30114, #100127 ) ;
#11340=DIRECTION ( 'NONE',  ( 0.000000000000000000, 1.000000000000000000, 0.000000000000000000 ) ) ;
#11341=DIRECTION ( 'NONE',  ( 0.000000000000000000, 1.000000000000000000, 0.000000000000000000 ) ) ;
#11342=DIRECTION ( 'NONE',  ( 0.000000000000000000, 1.000000000000000000, 0.000000000000000000 ) ) ;
#11343=FACE_OUTER_BOUND ( 'NONE', #31713, .T. ) ;
#11344=DIRECTION ( 'NONE',  ( 0.000000000000000000, 0.000000000000000000, 1.000000000000000000 ) ) ;
#11345=CARTESIAN_POINT ( 'NONE',  ( -14.14999999999998792, 2.500000000000000000, -1.472243186433547901 ) ) ;
#11346=CARTESIAN_POINT ( 'NONE',  ( -2.500000000000030642, 2.500000000000000000, -4.922947341949753586 ) ) ;
#11347=AXIS2_PLACEMENT_3D ( 'NONE', #17030, #56980, #96915 ) ;
#11348=CONICAL_SURFACE ( 'NONE', #9191, 0.1000000000000002554, 0.003490658503988666988 ) ;
#11349=ORIENTED_EDGE ( 'NONE', *, *, #24118, .F. ) ;
#11351=ORIENTED_EDGE ( 'NONE', *, *, #107308, .F. ) ;
#11352=CARTESIAN_POINT ( 'NONE',  ( 10.44999999999991047, 2.500000000000000000, -6.495190528383302464 ) ) ;
#11353=DIRECTION ( 'NONE',  ( -0.000000000000000000, -1.000000000000000000, -0.000000000000000000 ) ) ;
#11354=ORIENTED_EDGE ( 'NONE', *, *, #112253, .F. ) ;
#11355=DIRECTION ( 'NONE',  ( 0.000000000000000000, 0.000000000000000000, 1.000000000000000000 ) ) ;
#11356=LINE ( 'NONE', #91208, #77052 ) ;
#11357=EDGE_LOOP ( 'NONE', ( #81779, #83728 ) ) ;
#11358=AXIS2_PLACEMENT_3D ( 'NONE', #76912, #96528, #16673 ) ;
#11359=DIRECTION ( 'NONE',  ( 0.000000000000000000, 1.000000000000000000, 0.000000000000000000 ) ) ;
#11360=ORIENTED_EDGE ( 'NONE', *, *, #12512, .F. ) ;
#11361=ORIENTED_EDGE ( 'NONE', *, *, #6494, .F. ) ;
#11362=DIRECTION ( 'NONE',  ( 0.000000000000000000, 1.000000000000000000, 0.000000000000000000 ) ) ;
#11363=DIRECTION ( 'NONE',  ( 0.000000000000000000, -0.9999939076577903929, 0.003490651415223739937 ) ) ;
#11364=DIRECTION ( 'NONE',  ( 0.000000000000000000, 1.000000000000000000, 0.000000000000000000 ) ) ;
#11365=DIRECTION ( 'NONE',  ( 0.000000000000000000, 1.000000000000000000, 0.000000000000000000 ) ) ;
#11367=EDGE_CURVE ( 'NONE', #41239, #128359, #11074, .T. ) ;
#11368=VERTEX_POINT ( 'NONE', #52087 ) ;
#11369=CIRCLE ( 'NONE', #92857, 0.1000000000000000472 ) ;
#11370=LINE ( 'NONE', #72246, #61316 ) ;
#11371=AXIS2_PLACEMENT_3D ( 'NONE', #95647, #104800, #85812 ) ;
#11372=VERTEX_POINT ( 'NONE', #83487 ) ;
#11373=PLANE ( 'NONE',  #75820 ) ;
#11374=DIRECTION ( 'NONE',  ( 0.000000000000000000, 0.000000000000000000, 1.000000000000000000 ) ) ;
#11376=DIRECTION ( 'NONE',  ( 0.000000000000000000, -0.9999939076577903929, 0.003490651415223739937 ) ) ;
#11377=CARTESIAN_POINT ( 'NONE',  ( 6.049999999999934097, 2.500000000000000000, -2.411473670974877859 ) ) ;
#11378=CARTESIAN_POINT ( 'NONE',  ( -8.750000000000005329, 2.500000000000000000, 5.802370205355744659 ) ) ;
#11379=CARTESIAN_POINT ( 'NONE',  ( -6.450000000000019718, 12.50000000000000000, -1.818653347947326138 ) ) ;
#11382=CIRCLE ( 'NONE', #44851, 0.06509327318403745899 ) ;
#11383=DIRECTION ( 'NONE',  ( -0.000000000000000000, 1.000000000000000000, -0.000000000000000000 ) ) ;
#11384=DIRECTION ( 'NONE',  ( 0.000000000000000000, 1.000000000000000000, 0.000000000000000000 ) ) ;
#11385=CONICAL_SURFACE ( 'NONE', #61490, 0.1000000000000002554, 0.003490658503988666988 ) ;
#11386=AXIS2_PLACEMENT_3D ( 'NONE', #42931, #90711, #72375 ) ;
#11387=AXIS2_PLACEMENT_3D ( 'NONE', #81011, #69903, #60730 ) ;
#11388=ORIENTED_EDGE ( 'NONE', *, *, #125283, .F. ) ;
#11389=DIRECTION ( 'NONE',  ( 0.000000000000000000, 0.000000000000000000, -1.000000000000000000 ) ) ;
#11390=VECTOR ( 'NONE', #49671, 1000.000000000000000 ) ;
#11391=AXIS2_PLACEMENT_3D ( 'NONE', #39339, #38020, #19676 ) ;
#11392=EDGE_LOOP ( 'NONE', ( #76262, #36804 ) ) ;
#11393=CIRCLE ( 'NONE', #80369, 0.09999999999999982514 ) ;
#11394=EDGE_LOOP ( 'NONE', ( #54022, #22723, #25974, #80907 ) ) ;
#11395=LINE ( 'NONE', #51350, #55132 ) ;
#11397=CARTESIAN_POINT ( 'NONE',  ( -4.350000000000023626, 12.50000000000000000, 6.906693963081109722 ) ) ;
#11398=CARTESIAN_POINT ( 'NONE',  ( 3.949999999999938893, 2.500000000000000000, 6.148780366869520009 ) ) ;
#11399=CARTESIAN_POINT ( 'NONE',  ( 8.549999999999918998, 2.500000000000000000, 6.841600689897072485 ) ) ;
#11400=ORIENTED_EDGE ( 'NONE', *, *, #47219, .T. ) ;
#11401=AXIS2_PLACEMENT_3D ( 'NONE', #48376, #37280, #26803 ) ;
#11402=VECTOR ( 'NONE', #11759, 1000.000000000000000 ) ;
#11403=EDGE_CURVE ( 'NONE', #125479, #15328, #63838, .T. ) ;
#11404=DIRECTION ( 'NONE',  ( -0.000000000000000000, -1.000000000000000000, -0.000000000000000000 ) ) ;
#11405=CARTESIAN_POINT ( 'NONE',  ( 1.649999999999949729, 12.50000000000000000, 5.737276932171707422 ) ) ;
#11406=EDGE_CURVE ( 'NONE', #75500, #124247, #111427, .T. ) ;
#11407=EDGE_CURVE ( 'NONE', #74772, #59434, #36145, .T. ) ;
#11408=VERTEX_POINT ( 'NONE', #2309 ) ;
#11409=ORIENTED_EDGE ( 'NONE', *, *, #3712, .F. ) ;
#11410=EDGE_LOOP ( 'NONE', ( #122507, #33811 ) ) ;
#11411=DIRECTION ( 'NONE',  ( -0.000000000000000000, -1.000000000000000000, -0.000000000000000000 ) ) ;
#11413=ADVANCED_FACE ( 'NONE', ( #82845 ), #72376, .T. ) ;
#11414=EDGE_CURVE ( 'NONE', #28130, #91712, #59134, .T. ) ;
#11415=DIRECTION ( 'NONE',  ( -0.000000000000000000, -1.000000000000000000, -0.000000000000000000 ) ) ;
#11416=EDGE_CURVE ( 'NONE', #16149, #29869, #23247, .T. ) ;
#11417=FACE_BOUND ( 'NONE', #27345, .T. ) ;
#11418=ORIENTED_EDGE ( 'NONE', *, *, #13818, .T. ) ;
#11419=EDGE_CURVE ( 'NONE', #78711, #75943, #41641, .T. ) ;
#11420=EDGE_CURVE ( 'NONE', #52365, #119493, #12776, .T. ) ;
#11421=DIRECTION ( 'NONE',  ( 0.000000000000000000, 0.000000000000000000, -1.000000000000000000 ) ) ;
#11422=CARTESIAN_POINT ( 'NONE',  ( 14.14999999999989733, 2.500000000000000000, 2.857883832488649301 ) ) ;
#11423=AXIS2_PLACEMENT_3D ( 'NONE', #80911, #53228, #58689 ) ;
#11424=ORIENTED_EDGE ( 'NONE', *, *, #50622, .F. ) ;
#11425=PLANE ( 'NONE',  #57197 ) ;
#11426=DIRECTION ( 'NONE',  ( 0.000000000000000000, 1.000000000000000000, 0.000000000000000000 ) ) ;
#11427=CARTESIAN_POINT ( 'NONE',  ( -11.69999999999999929, 12.50000000000000000, 1.734723475976807094E-15 ) ) ;
#11428=DIRECTION ( 'NONE',  ( 0.000000000000000000, 0.000000000000000000, -1.000000000000000000 ) ) ;
#11429=DIRECTION ( 'NONE',  ( -4.274815082592931898E-19, -0.9999939076577903929, -0.003490651415223739937 ) ) ;
#11430=EDGE_CURVE ( 'NONE', #126385, #119822, #71740, .T. ) ;
#11431=DIRECTION ( 'NONE',  ( 0.000000000000000000, -0.9999939076577903929, 0.003490651415223739937 ) ) ;
#11432=DIRECTION ( 'NONE',  ( -0.000000000000000000, -1.000000000000000000, -0.000000000000000000 ) ) ;
#11433=AXIS2_PLACEMENT_3D ( 'NONE', #121546, #122853, #51550 ) ;
#11434=CONICAL_SURFACE ( 'NONE', #84603, 0.1000000000000000056, 0.003490658503988666988 ) ;
#11435=ORIENTED_EDGE ( 'NONE', *, *, #120967, .F. ) ;
#11436=ORIENTED_EDGE ( 'NONE', *, *, #109832, .T. ) ;
#11437=VERTEX_POINT ( 'NONE', #113577 ) ;
#11438=EDGE_LOOP ( 'NONE', ( #100150, #46702 ) ) ;
#11439=DIRECTION ( 'NONE',  ( 0.000000000000000000, -0.000000000000000000, 1.000000000000000000 ) ) ;
#11440=DIRECTION ( 'NONE',  ( 0.000000000000000000, -0.9999939076577903929, 0.003490651415223739937 ) ) ;
#11441=ORIENTED_EDGE ( 'NONE', *, *, #54994, .F. ) ;
#11442=FACE_BOUND ( 'NONE', #84999, .T. ) ;
#11443=DIRECTION ( 'NONE',  ( 0.000000000000000000, -0.000000000000000000, 1.000000000000000000 ) ) ;
#11444=DIRECTION ( 'NONE',  ( 0.000000000000000000, 0.000000000000000000, 1.000000000000000000 ) ) ;
#11445=CIRCLE ( 'NONE', #44906, 0.06509327318403745899 ) ;
#11446=DIRECTION ( 'NONE',  ( -0.000000000000000000, -1.000000000000000000, -0.000000000000000000 ) ) ;
#11447=DIRECTION ( 'NONE',  ( 0.000000000000000000, 0.000000000000000000, 1.000000000000000000 ) ) ;
#11449=CARTESIAN_POINT ( 'NONE',  ( -4.150000000000027889, 12.50000000000000000, -7.122917578226816815 ) ) ;
#11450=DIRECTION ( 'NONE',  ( 0.000000000000000000, -0.000000000000000000, 1.000000000000000000 ) ) ;
#11451=LINE ( 'NONE', #120766, #53829 ) ;
#11452=CARTESIAN_POINT ( 'NONE',  ( -1.450000000000035927, 2.500000000000000000, -6.048780366869526581 ) ) ;
#11453=DIRECTION ( 'NONE',  ( -4.274815082592931898E-19, -0.9999939076577903929, -0.003490651415223739937 ) ) ;
#11454=ORIENTED_EDGE ( 'NONE', *, *, #121383, .T. ) ;
#11455=EDGE_LOOP ( 'NONE', ( #35355, #87114 ) ) ;
#11456=AXIS2_PLACEMENT_3D ( 'NONE', #28820, #68078, #108650 ) ;
#11457=ORIENTED_EDGE ( 'NONE', *, *, #110973, .T. ) ;
#11458=VERTEX_POINT ( 'NONE', #88945 ) ;
#11459=AXIS2_PLACEMENT_3D ( 'NONE', #88044, #39652, #68430 ) ;
#11460=VERTEX_POINT ( 'NONE', #53377 ) ;
#11461=EDGE_LOOP ( 'NONE', ( #65054, #48773, #28101, #102716 ) ) ;
#11462=CARTESIAN_POINT ( 'NONE',  ( -7.700000000000012612, 2.500000000000000000, 4.576537180435972019 ) ) ;
#11463=EDGE_CURVE ( 'NONE', #65404, #126067, #71638, .T. ) ;
#11464=VERTEX_POINT ( 'NONE', #49038 ) ;
#11465=EDGE_CURVE ( 'NONE', #10941, #44142, #93291, .T. ) ;
#11466=CONICAL_SURFACE ( 'NONE', #88742, 0.09999999999999999167, 0.003490658503988666988 ) ;
#11468=CARTESIAN_POINT ( 'NONE',  ( 16.70850060796067993, 0.4765610498145415042, 5.930927070179838445 ) ) ;
#11469=PLANE ( 'NONE',  #122789 ) ;
#11470=DIRECTION ( 'NONE',  ( -0.000000000000000000, -1.000000000000000000, -0.000000000000000000 ) ) ;
#11471=DIRECTION ( 'NONE',  ( 0.000000000000000000, 0.000000000000000000, 1.000000000000000000 ) ) ;
#11472=ADVANCED_FACE ( 'NONE', ( #62555 ), #82103, .T. ) ;
#11473=ORIENTED_EDGE ( 'NONE', *, *, #68314, .F. ) ;
#11474=LINE ( 'NONE', #112268, #8783 ) ;
#11475=ADVANCED_FACE ( 'NONE', ( #23916 ), #13127, .T. ) ;
#11476=EDGE_CURVE ( 'NONE', #67419, #82776, #89588, .T. ) ;
#11477=ORIENTED_EDGE ( 'NONE', *, *, #24456, .F. ) ;
#11478=EDGE_CURVE ( 'NONE', #80386, #99444, #109288, .T. ) ;
#11479=CONICAL_SURFACE ( 'NONE', #99227, 0.1000000000000002554, 0.003490658503988666988 ) ;
#11480=ORIENTED_EDGE ( 'NONE', *, *, #108097, .F. ) ;
#11482=AXIS2_PLACEMENT_3D ( 'NONE', #102480, #71086, #121459 ) ;
#11483=DIRECTION ( 'NONE',  ( 0.000000000000000000, 1.000000000000000000, 0.000000000000000000 ) ) ;
#11484=AXIS2_PLACEMENT_3D ( 'NONE', #99862, #102900, #9544 ) ;
#11485=DIRECTION ( 'NONE',  ( -0.000000000000000000, -1.000000000000000000, -0.000000000000000000 ) ) ;
#11486=ORIENTED_EDGE ( 'NONE', *, *, #44884, .T. ) ;
#11487=EDGE_CURVE ( 'NONE', #24791, #45310, #126001, .T. ) ;
#11488=ORIENTED_EDGE ( 'NONE', *, *, #17164, .F. ) ;
#11489=CARTESIAN_POINT ( 'NONE',  ( -1.050000000000037348, 2.500000000000000000, -2.511473670974877948 ) ) ;
#11490=CIRCLE ( 'NONE', #59639, 0.06509327318403745899 ) ;
#11491=AXIS2_PLACEMENT_3D ( 'NONE', #47053, #86963, #24185 ) ;
#11492=CONICAL_SURFACE ( 'NONE', #128600, 0.1000000000000002554, 0.003490658503988666988 ) ;
#11493=LINE ( 'NONE', #51438, #118509 ) ;
#11495=DIRECTION ( 'NONE',  ( -0.000000000000000000, -1.000000000000000000, -0.000000000000000000 ) ) ;
#11496=EDGE_LOOP ( 'NONE', ( #112391, #101191, #55332, #68630 ) ) ;
#11497=CIRCLE ( 'NONE', #36654, 0.1000000000000002554 ) ;
#11498=CARTESIAN_POINT ( 'NONE',  ( -10.85000000000000142, 2.500000000000000000, 6.595190528383296780 ) ) ;
#11499=ORIENTED_EDGE ( 'NONE', *, *, #94951, .T. ) ;
#11500=LINE ( 'NONE', #22629, #59452 ) ;
#11501=AXIS2_PLACEMENT_3D ( 'NONE', #42209, #82787, #103707 ) ;
#11502=EDGE_LOOP ( 'NONE', ( #87579, #70359, #27440, #63042 ) ) ;
#11503=FACE_OUTER_BOUND ( 'NONE', #5142, .T. ) ;
#11504=LINE ( 'NONE', #110970, #10794 ) ;
#11505=CARTESIAN_POINT ( 'NONE',  ( -10.40000000000000213, 2.500000000000000000, 4.922947341949748257 ) ) ;
#11506=AXIS2_PLACEMENT_3D ( 'NONE', #20707, #41016, #98592 ) ;
#11507=EDGE_CURVE ( 'NONE', #37844, #93665, #65459, .T. ) ;
#11508=DIRECTION ( 'NONE',  ( 0.000000000000000000, 0.000000000000000000, -1.000000000000000000 ) ) ;
#11509=VERTEX_POINT ( 'NONE', #46779 ) ;
#11510=CARTESIAN_POINT ( 'NONE',  ( -3.950000000000026379, 2.500000000000000000, 6.741600689897071952 ) ) ;
#11511=DIRECTION ( 'NONE',  ( 0.000000000000000000, 1.000000000000000000, 0.000000000000000000 ) ) ;
#11512=VERTEX_POINT ( 'NONE', #27133 ) ;
#11513=VERTEX_POINT ( 'NONE', #75573 ) ;
#11514=EDGE_LOOP ( 'NONE', ( #73506, #37314, #64802, #114939 ) ) ;
#11515=CARTESIAN_POINT ( 'NONE',  ( 17.50000000000000000, 2.750000000000000000, 2.864912725862981624 ) ) ;
#11516=DIRECTION ( 'NONE',  ( -0.000000000000000000, -1.000000000000000000, -0.000000000000000000 ) ) ;
#11518=AXIS2_PLACEMENT_3D ( 'NONE', #119956, #51235, #121241 ) ;
#11519=CARTESIAN_POINT ( 'NONE',  ( 12.89999999999990266, 12.50000000000000000, 3.572213422710607489 ) ) ;
#11520=DIRECTION ( 'NONE',  ( -0.000000000000000000, 1.000000000000000000, -0.000000000000000000 ) ) ;
#11521=DIRECTION ( 'NONE',  ( 0.000000000000000000, 0.000000000000000000, -1.000000000000000000 ) ) ;
#11522=EDGE_CURVE ( 'NONE', #59844, #74070, #103127, .T. ) ;
#11523=DIRECTION ( 'NONE',  ( -0.000000000000000000, 1.000000000000000000, -0.000000000000000000 ) ) ;
#11524=DIRECTION ( 'NONE',  ( 0.000000000000000000, -0.000000000000000000, 1.000000000000000000 ) ) ;
#11525=CONICAL_SURFACE ( 'NONE', #24057, 0.1000000000000000472, 0.003490658503988666988 ) ;
#11526=CIRCLE ( 'NONE', #9475, 0.06509327318403745899 ) ;
#11527=VERTEX_POINT ( 'NONE', #34393 ) ;
#11528=CARTESIAN_POINT ( 'NONE',  ( -7.950000000000016165, 2.500000000000000000, -6.495190528383297135 ) ) ;
#11529=ADVANCED_FACE ( 'NONE', ( #104401 ), #116144, .T. ) ;
#11530=DIRECTION ( 'NONE',  ( -0.000000000000000000, -1.000000000000000000, -0.000000000000000000 ) ) ;
#11531=LINE ( 'NONE', #61289, #33861 ) ;
#11532=CARTESIAN_POINT ( 'NONE',  ( -7.900000000000011013, 2.500000000000000000, 3.737306695894644371 ) ) ;
#11533=VERTEX_POINT ( 'NONE', #15349 ) ;
#11534=CARTESIAN_POINT ( 'NONE',  ( 5.599999999999934808, 2.500000000000000000, -3.983716857408426293 ) ) ;
#11535=CIRCLE ( 'NONE', #47143, 0.1000000000000000056 ) ;
#11536=AXIS2_PLACEMENT_3D ( 'NONE', #29477, #9829, #102705 ) ;
#11537=CARTESIAN_POINT ( 'NONE',  ( 8.549999999999920774, 2.500000000000000000, -2.511473670974877948 ) ) ;
#11538=DIRECTION ( 'NONE',  ( -0.000000000000000000, 1.000000000000000000, -0.000000000000000000 ) ) ;
#11540=ORIENTED_EDGE ( 'NONE', *, *, #62244, .F. ) ;
#11541=DIRECTION ( 'NONE',  ( -0.000000000000000000, 1.000000000000000000, -0.000000000000000000 ) ) ;
#11542=AXIS2_PLACEMENT_3D ( 'NONE', #28501, #88702, #129299 ) ;
#11543=ORIENTED_EDGE ( 'NONE', *, *, #55131, .F. ) ;
#11544=EDGE_LOOP ( 'NONE', ( #124246, #124825, #113784, #3602 ) ) ;
#11545=DIRECTION ( 'NONE',  ( 0.000000000000000000, 0.000000000000000000, -1.000000000000000000 ) ) ;
#11546=CARTESIAN_POINT ( 'NONE',  ( 3.149999999999946176, 2.500000000000000000, -6.148780366869526226 ) ) ;
#11547=DIRECTION ( 'NONE',  ( -0.000000000000000000, -1.000000000000000000, -0.000000000000000000 ) ) ;
#11548=CARTESIAN_POINT ( 'NONE',  ( 15.83209681635555022, 2.500000000000000000, -5.404881881984143099 ) ) ;
#11549=ORIENTED_EDGE ( 'NONE', *, *, #37870, .T. ) ;
#11550=ADVANCED_FACE ( 'NONE', ( #6181 ), #67602, .T. ) ;
#11551=DIRECTION ( 'NONE',  ( -0.000000000000000000, 1.000000000000000000, -0.000000000000000000 ) ) ;
#11552=ORIENTED_EDGE ( 'NONE', *, *, #107469, .T. ) ;
#11553=CARTESIAN_POINT ( 'NONE',  ( 17.50000000000010658, 2.362777783882526350, 3.757134105503078469 ) ) ;
#11554=DIRECTION ( 'NONE',  ( -0.000000000000000000, -1.000000000000000000, -0.000000000000000000 ) ) ;
#11555=AXIS2_PLACEMENT_3D ( 'NONE', #1341, #111278, #30184 ) ;
#11556=ADVANCED_FACE ( 'NONE', ( #125330 ), #25756, .T. ) ;
#11557=ORIENTED_EDGE ( 'NONE', *, *, #21654, .T. ) ;
#11558=CIRCLE ( 'NONE', #93057, 0.06509327318403745899 ) ;
#11559=EDGE_LOOP ( 'NONE', ( #4061, #6503 ) ) ;
#11560=CIRCLE ( 'NONE', #26157, 0.09999999999999982514 ) ;
#11561=ORIENTED_EDGE ( 'NONE', *, *, #51653, .T. ) ;
#11562=ORIENTED_EDGE ( 'NONE', *, *, #128317, .T. ) ;
#11563=CARTESIAN_POINT ( 'NONE',  ( -13.09999999999999254, 2.500000000000000000, -4.676537180435975216 ) ) ;
#11564=DIRECTION ( 'NONE',  ( 0.000000000000000000, 0.000000000000000000, 1.000000000000000000 ) ) ;
#11565=EDGE_CURVE ( 'NONE', #18996, #102121, #95233, .T. ) ;
#11566=CIRCLE ( 'NONE', #26159, 0.09999999999999999167 ) ;
#11567=EDGE_CURVE ( 'NONE', #70253, #113534, #36237, .T. ) ;
#11568=DIRECTION ( 'NONE',  ( 0.000000000000000000, 1.000000000000000000, 0.000000000000000000 ) ) ;
#11569=EDGE_CURVE ( 'NONE', #63649, #13514, #82205, .T. ) ;
#11570=FACE_BOUND ( 'NONE', #24913, .T. ) ;
#11571=ADVANCED_FACE ( 'NONE', ( #4243 ), #44182, .T. ) ;
#11572=CARTESIAN_POINT ( 'NONE',  ( 1.249999999999988898, 12.50000000000000000, -6.495190528383302464 ) ) ;
#11574=DIRECTION ( 'NONE',  ( 0.000000000000000000, 0.000000000000000000, 1.000000000000000000 ) ) ;
#11575=CARTESIAN_POINT ( 'NONE',  ( -5.800000000000022027, 12.50000000000000000, -4.395220292106239768 ) ) ;
#11576=CONICAL_SURFACE ( 'NONE', #84739, 0.09999999999999982514, 0.003490658503988666988 ) ;
#11577=CIRCLE ( 'NONE', #95214, 0.06509327318403745899 ) ;
#11578=CARTESIAN_POINT ( 'NONE',  ( 12.69999999999990337, 2.500000000000000000, 4.083716857408420609 ) ) ;
#11579=CIRCLE ( 'NONE', #45054, 0.09999999999999982514 ) ;
#11580=DIRECTION ( 'NONE',  ( 0.000000000000000000, 1.000000000000000000, 0.000000000000000000 ) ) ;
#11581=ADVANCED_FACE ( 'NONE', ( #24548 ), #46692, .T. ) ;
#11582=CARTESIAN_POINT ( 'NONE',  ( 1.249999999999952038, 2.500000000000000000, 5.802370205355744659 ) ) ;
#11583=EDGE_CURVE ( 'NONE', #19309, #65281, #88445, .T. ) ;
#11584=CIRCLE ( 'NONE', #128701, 0.06509327318403745899 ) ;
#11585=AXIS2_PLACEMENT_3D ( 'NONE', #72802, #13861, #43993 ) ;
#11586=EDGE_CURVE ( 'NONE', #54506, #102089, #48759, .T. ) ;
#11587=CARTESIAN_POINT ( 'NONE',  ( 14.14999999999989377, 2.500000000000000000, -1.472243186433550122 ) ) ;
#11588=CIRCLE ( 'NONE', #47195, 0.1000000000000002554 ) ;
#11589=ORIENTED_EDGE ( 'NONE', *, *, #80662, .T. ) ;
#11590=ORIENTED_EDGE ( 'NONE', *, *, #50560, .T. ) ;
#11591=ORIENTED_EDGE ( 'NONE', *, *, #123570, .F. ) ;
#11592=VERTEX_POINT ( 'NONE', #45496 ) ;
#11593=VECTOR ( 'NONE', #94923, 1000.000000000000000 ) ;
#11595=DIRECTION ( 'NONE',  ( 0.000000000000000000, 0.000000000000000000, -1.000000000000000000 ) ) ;
#11596=DIRECTION ( 'NONE',  ( -0.000000000000000000, -1.000000000000000000, -0.000000000000000000 ) ) ;
#11597=ORIENTED_EDGE ( 'NONE', *, *, #65200, .F. ) ;
#11598=FACE_BOUND ( 'NONE', #58262, .T. ) ;
#11599=CARTESIAN_POINT ( 'NONE',  ( 0.3999999999999559464, 2.500000000000000000, -4.330127018922201643 ) ) ;
#11600=VERTEX_POINT ( 'NONE', #86023 ) ;
#11601=CARTESIAN_POINT ( 'NONE',  ( 8.749999999999921840, 2.500000000000000000, 2.857883832488649301 ) ) ;
#11602=DIRECTION ( 'NONE',  ( -0.000000000000000000, 1.000000000000000000, -0.000000000000000000 ) ) ;
#11603=DIRECTION ( 'NONE',  ( 0.000000000000000000, 0.000000000000000000, -1.000000000000000000 ) ) ;
#11604=DIRECTION ( 'NONE',  ( 0.000000000000000000, 1.000000000000000000, 0.000000000000000000 ) ) ;
#11605=CIRCLE ( 'NONE', #49285, 0.1000000000000002554 ) ;
#11606=ORIENTED_EDGE ( 'NONE', *, *, #90779, .T. ) ;
#11607=DIRECTION ( 'NONE',  ( 0.000000000000000000, 0.000000000000000000, -1.000000000000000000 ) ) ;
#11608=EDGE_LOOP ( 'NONE', ( #32035, #59023, #125745, #24689 ) ) ;
#11609=EDGE_LOOP ( 'NONE', ( #62790, #72339, #104159, #19984 ) ) ;
#11610=DIRECTION ( 'NONE',  ( 0.000000000000000000, 1.000000000000000000, 0.000000000000000000 ) ) ;
#11611=LINE ( 'NONE', #112404, #74814 ) ;
#11612=AXIS2_PLACEMENT_3D ( 'NONE', #62970, #82627, #21107 ) ;
#11613=EDGE_LOOP ( 'NONE', ( #112554, #88040 ) ) ;
#11614=DIRECTION ( 'NONE',  ( 0.000000000000000000, 1.000000000000000000, 0.000000000000000000 ) ) ;
#11615=AXIS2_PLACEMENT_3D ( 'NONE', #12069, #82771, #4167 ) ;
#11616=AXIS2_PLACEMENT_3D ( 'NONE', #88706, #99179, #38331 ) ;
#11617=DIRECTION ( 'NONE',  ( 0.000000000000000000, 0.000000000000000000, -1.000000000000000000 ) ) ;
#11618=CARTESIAN_POINT ( 'NONE',  ( 3.949999999999938893, 2.500000000000000000, 6.148780366869520009 ) ) ;
#11619=DIRECTION ( 'NONE',  ( 0.000000000000000000, 1.000000000000000000, 0.000000000000000000 ) ) ;
#11620=DIRECTION ( 'NONE',  ( -4.274815082592931898E-19, -0.9999939076577903929, -0.003490651415223739937 ) ) ;
#11621=EDGE_LOOP ( 'NONE', ( #95465, #12397, #28165, #85984 ) ) ;
#11622=FACE_OUTER_BOUND ( 'NONE', #121884, .T. ) ;
#11623=EDGE_CURVE ( 'NONE', #88605, #56169, #128277, .T. ) ;
#11624=VERTEX_POINT ( 'NONE', #76238 ) ;
#11625=DIRECTION ( 'NONE',  ( 0.000000000000000000, 1.000000000000000000, 0.000000000000000000 ) ) ;
#11626=AXIS2_PLACEMENT_3D ( 'NONE', #13651, #14295, #102679 ) ;
#11627=EDGE_CURVE ( 'NONE', #26724, #113868, #113596, .T. ) ;
#11628=ORIENTED_EDGE ( 'NONE', *, *, #90273, .F. ) ;
#11629=CIRCLE ( 'NONE', #15831, 0.09999999999999999167 ) ;
#11630=LINE ( 'NONE', #50926, #39296 ) ;
#11631=EDGE_CURVE ( 'NONE', #8603, #93230, #80145, .T. ) ;
#11632=ORIENTED_EDGE ( 'NONE', *, *, #24080, .F. ) ;
#11633=CARTESIAN_POINT ( 'NONE',  ( -8.300000000000011369, 2.500000000000000000, -2.276824562219559311E-15 ) ) ;
#11634=DIRECTION ( 'NONE',  ( -0.000000000000000000, 1.000000000000000000, -0.000000000000000000 ) ) ;
#11635=DIRECTION ( 'NONE',  ( 0.000000000000000000, 1.000000000000000000, 0.000000000000000000 ) ) ;
#11636=DIRECTION ( 'NONE',  ( 0.000000000000000000, 0.000000000000000000, 1.000000000000000000 ) ) ;
#11638=EDGE_LOOP ( 'NONE', ( #65945, #88227 ) ) ;
#11639=EDGE_CURVE ( 'NONE', #26161, #102161, #15266, .T. ) ;
#11640=VERTEX_POINT ( 'NONE', #54638 ) ;
#11641=ORIENTED_EDGE ( 'NONE', *, *, #7715, .T. ) ;
#11642=PLANE ( 'NONE',  #80958 ) ;
#11643=AXIS2_PLACEMENT_3D ( 'NONE', #89827, #57805, #90460 ) ;
#11644=CARTESIAN_POINT ( 'NONE',  ( -7.500000000000011546, 2.500000000000000000, 3.737306695894644371 ) ) ;
#11645=CARTESIAN_POINT ( 'NONE',  ( 2.099999999999950351, 2.500000000000000000, -5.022947341949754119 ) ) ;
#11646=ORIENTED_EDGE ( 'NONE', *, *, #40896, .T. ) ;
#11647=ORIENTED_EDGE ( 'NONE', *, *, #35434, .T. ) ;
#11648=ORIENTED_EDGE ( 'NONE', *, *, #70288, .T. ) ;
#11649=PLANE ( 'NONE',  #85451 ) ;
#11650=ORIENTED_EDGE ( 'NONE', *, *, #80000, .T. ) ;
#11651=CARTESIAN_POINT ( 'NONE',  ( 6.649999999999930189, 2.500000000000000000, -1.472243186433550122 ) ) ;
#11652=FACE_OUTER_BOUND ( 'NONE', #103116, .T. ) ;
#11653=CARTESIAN_POINT ( 'NONE',  ( -10.85000000000000142, 2.500000000000000000, -5.902370205355746968 ) ) ;
#11654=DIRECTION ( 'NONE',  ( 0.000000000000000000, 0.000000000000000000, -1.000000000000000000 ) ) ;
#11656=CARTESIAN_POINT ( 'NONE',  ( 7.299999999999924327, 2.500000000000000000, 0.3464101615137735735 ) ) ;
#11657=FACE_OUTER_BOUND ( 'NONE', #23066, .T. ) ;
#11658=EDGE_CURVE ( 'NONE', #108389, #96060, #87955, .T. ) ;
#11659=CARTESIAN_POINT ( 'NONE',  ( 3.949999999999938005, 2.500000000000000000, 6.841600689897072485 ) ) ;
#11660=ORIENTED_EDGE ( 'NONE', *, *, #98655, .F. ) ;
#11661=DIRECTION ( 'NONE',  ( -0.000000000000000000, 1.000000000000000000, -0.000000000000000000 ) ) ;
#11662=AXIS2_PLACEMENT_3D ( 'NONE', #114798, #74243, #112881 ) ;
#11663=AXIS2_PLACEMENT_3D ( 'NONE', #32966, #100399, #10693 ) ;
#11664=DIRECTION ( 'NONE',  ( 0.000000000000000000, -0.9999939076577903929, 0.003490651415223739937 ) ) ;
#11665=ORIENTED_EDGE ( 'NONE', *, *, #93777, .T. ) ;
#11666=ORIENTED_EDGE ( 'NONE', *, *, #11420, .F. ) ;
#11668=DIRECTION ( 'NONE',  ( 0.000000000000000000, 0.000000000000000000, -1.000000000000000000 ) ) ;
#11669=DIRECTION ( 'NONE',  ( 0.000000000000000000, -0.9999939076577903929, 0.003490651415223739937 ) ) ;
#11670=CARTESIAN_POINT ( 'NONE',  ( 1.699999999999951994, 12.50000000000000000, -4.330127018922201643 ) ) ;
#11671=CARTESIAN_POINT ( 'NONE',  ( 13.74999999999989697, 12.50000000000000000, 2.857883832488649301 ) ) ;
#11672=DIRECTION ( 'NONE',  ( 0.000000000000000000, 0.000000000000000000, 1.000000000000000000 ) ) ;
#11673=ADVANCED_FACE ( 'NONE', ( #127275 ), #21659, .T. ) ;
#11674=CARTESIAN_POINT ( 'NONE',  ( 9.599999999999917932, 12.50000000000000000, 0.6277270498435120194 ) ) ;
#11675=CARTESIAN_POINT ( 'NONE',  ( 4.549999999999939426, 2.500000000000000000, -6.395190528383301931 ) ) ;
#11676=AXIS2_PLACEMENT_3D ( 'NONE', #46812, #7513, #47453 ) ;
#11677=CARTESIAN_POINT ( 'NONE',  ( -12.89999999999999147, 2.500000000000000000, -4.922947341949750921 ) ) ;
#11678=AXIS2_PLACEMENT_3D ( 'NONE', #95884, #18605, #68348 ) ;
#11679=AXIS2_PLACEMENT_3D ( 'NONE', #98220, #8537, #48487 ) ;
#11680=ORIENTED_EDGE ( 'NONE', *, *, #35929, .F. ) ;
#11681=VERTEX_POINT ( 'NONE', #79465 ) ;
#11682=AXIS2_PLACEMENT_3D ( 'NONE', #50441, #71357, #49185 ) ;
#11684=CIRCLE ( 'NONE', #128503, 0.06509327318403743123 ) ;
#11685=EDGE_LOOP ( 'NONE', ( #127081, #66376, #81529, #44408 ) ) ;
#11686=EDGE_CURVE ( 'NONE', #73744, #115596, #108260, .T. ) ;
#11687=CARTESIAN_POINT ( 'NONE',  ( -0.8500000000000382805, 2.500000000000000000, -5.802370205355749988 ) ) ;
#11688=CARTESIAN_POINT ( 'NONE',  ( 7.499999999999961808, 12.50000000000000000, 4.330127018922196314 ) ) ;
#11689=ORIENTED_EDGE ( 'NONE', *, *, #13497, .F. ) ;
#11690=DIRECTION ( 'NONE',  ( -0.000000000000000000, -1.000000000000000000, -0.000000000000000000 ) ) ;
#11691=DIRECTION ( 'NONE',  ( -0.000000000000000000, -1.000000000000000000, -0.000000000000000000 ) ) ;
#11692=CARTESIAN_POINT ( 'NONE',  ( -3.644143946350442628E-14, 2.500000000000000000, 0.5928203230275517210 ) ) ;
#11694=ORIENTED_EDGE ( 'NONE', *, *, #126365, .T. ) ;
#11695=EDGE_CURVE ( 'NONE', #17926, #90702, #124052, .T. ) ;
#11696=CARTESIAN_POINT ( 'NONE',  ( 6.649999999999930189, 12.50000000000000000, 7.188010851410848723 ) ) ;
#11697=VECTOR ( 'NONE', #57509, 1000.000000000000000 ) ;
#11698=DIRECTION ( 'NONE',  ( -0.000000000000000000, 1.000000000000000000, -0.000000000000000000 ) ) ;
#11699=VERTEX_POINT ( 'NONE', #229 ) ;
#11700=ORIENTED_EDGE ( 'NONE', *, *, #40467, .F. ) ;
#11701=VERTEX_POINT ( 'NONE', #17275 ) ;
#11702=VERTEX_POINT ( 'NONE', #48068 ) ;
#11703=LINE ( 'NONE', #100098, #65598 ) ;
#11704=CIRCLE ( 'NONE', #74406, 0.1000000000000000056 ) ;
#11705=VECTOR ( 'NONE', #72777, 1000.000000000000000 ) ;
#11706=FACE_OUTER_BOUND ( 'NONE', #31501, .T. ) ;
#11707=CARTESIAN_POINT ( 'NONE',  ( 2.500000000000002220, -2.500000000000000000, -8.999999999999998224 ) ) ;
#11708=AXIS2_PLACEMENT_3D ( 'NONE', #84025, #85324, #93861 ) ;
#11709=VERTEX_POINT ( 'NONE', #87321 ) ;
#11710=CIRCLE ( 'NONE', #68141, 0.09999999999999999167 ) ;
#11711=EDGE_CURVE ( 'NONE', #24007, #127312, #101068, .T. ) ;
#11712=DIRECTION ( 'NONE',  ( 0.000000000000000000, -0.000000000000000000, 1.000000000000000000 ) ) ;
#11714=DIRECTION ( 'NONE',  ( 0.000000000000000000, 0.000000000000000000, 1.000000000000000000 ) ) ;
#11715=DIRECTION ( 'NONE',  ( 0.000000000000000000, -0.9999939076577903929, 0.003490651415223739937 ) ) ;
#11716=DIRECTION ( 'NONE',  ( -0.000000000000000000, -1.000000000000000000, -0.000000000000000000 ) ) ;
#11717=CARTESIAN_POINT ( 'NONE',  ( 0.3999999999999628852, 2.500000000000000000, 0.6928203230275518099 ) ) ;
#11718=AXIS2_PLACEMENT_3D ( 'NONE', #32041, #73236, #116999 ) ;
#11719=EDGE_CURVE ( 'NONE', #73752, #114231, #4909, .T. ) ;
#11720=ORIENTED_EDGE ( 'NONE', *, *, #50620, .F. ) ;
#11721=CONICAL_SURFACE ( 'NONE', #84880, 0.1000000000000002554, 0.003490658503988666988 ) ;
#11722=ORIENTED_EDGE ( 'NONE', *, *, #24321, .F. ) ;
#11724=CARTESIAN_POINT ( 'NONE',  ( -13.14999999999999147, 12.50000000000000000, -2.511473670974875727 ) ) ;
#11725=ADVANCED_FACE ( 'NONE', ( #117409 ), #59232, .T. ) ;
#11726=EDGE_CURVE ( 'NONE', #101017, #97372, #126103, .T. ) ;
#11727=DIRECTION ( 'NONE',  ( 0.000000000000000000, 0.000000000000000000, -1.000000000000000000 ) ) ;
#11729=FACE_BOUND ( 'NONE', #6724, .T. ) ;
#11730=ADVANCED_FACE ( 'NONE', ( #120025 ), #61367, .T. ) ;
#11731=FACE_OUTER_BOUND ( 'NONE', #15787, .T. ) ;
#11732=CARTESIAN_POINT ( 'NONE',  ( -10.40000000000000213, 2.500000000000000000, -4.922947341949749145 ) ) ;
#11733=DIRECTION ( 'NONE',  ( 0.000000000000000000, 1.000000000000000000, 0.000000000000000000 ) ) ;
#11734=EDGE_CURVE ( 'NONE', #56626, #40907, #92665, .T. ) ;
#11735=PLANE ( 'NONE',  #96504 ) ;
#11736=ADVANCED_FACE ( 'NONE', ( #109561 ), #38398, .T. ) ;
#11737=DIRECTION ( 'NONE',  ( -0.000000000000000000, 1.000000000000000000, -0.000000000000000000 ) ) ;
#11738=EDGE_CURVE ( 'NONE', #93976, #91980, #15367, .T. ) ;
#11739=CARTESIAN_POINT ( 'NONE',  ( 3.149999999999946176, 2.500000000000000000, -2.511473670974877948 ) ) ;
#11740=VERTEX_POINT ( 'NONE', #106961 ) ;
#11741=CARTESIAN_POINT ( 'NONE',  ( -7.300000000000013145, 2.500000000000000000, 3.883716857408420431 ) ) ;
#11742=EDGE_CURVE ( 'NONE', #64939, #28650, #32046, .T. ) ;
#11743=EDGE_CURVE ( 'NONE', #68741, #81973, #97798, .T. ) ;
#11744=DIRECTION ( 'NONE',  ( 0.000000000000000000, 0.000000000000000000, 1.000000000000000000 ) ) ;
#11745=ORIENTED_EDGE ( 'NONE', *, *, #22526, .F. ) ;
#11746=EDGE_LOOP ( 'NONE', ( #106242, #93809 ) ) ;
#11747=CARTESIAN_POINT ( 'NONE',  ( 5.599999999999931255, 2.500000000000000000, 4.676537180435972552 ) ) ;
#11748=ADVANCED_FACE ( 'NONE', ( #99748 ), #65562, .T. ) ;
#11749=DIRECTION ( 'NONE',  ( -0.000000000000000000, 1.000000000000000000, -0.000000000000000000 ) ) ;
#11750=FACE_BOUND ( 'NONE', #28613, .T. ) ;
#11751=ADVANCED_FACE ( 'NONE', ( #59184 ), #40549, .T. ) ;
#11752=LINE ( 'NONE', #89672, #53493 ) ;
#11753=AXIS2_PLACEMENT_3D ( 'NONE', #74099, #94364, #15801 ) ;
#11754=CONICAL_SURFACE ( 'NONE', #84915, 0.1000000000000002554, 0.003490658503988666988 ) ;
#11755=ORIENTED_EDGE ( 'NONE', *, *, #35621, .F. ) ;
#11756=DIRECTION ( 'NONE',  ( 0.000000000000000000, 1.000000000000000000, 0.000000000000000000 ) ) ;
#11757=DIRECTION ( 'NONE',  ( -0.000000000000000000, 1.000000000000000000, -0.000000000000000000 ) ) ;
#11759=DIRECTION ( 'NONE',  ( 0.000000000000000000, -0.9999939076577903929, 0.003490651415223739937 ) ) ;
#11760=DIRECTION ( 'NONE',  ( 0.000000000000000000, -0.000000000000000000, 1.000000000000000000 ) ) ;
#11761=CIRCLE ( 'NONE', #84923, 0.1000000000000002554 ) ;
#11762=CARTESIAN_POINT ( 'NONE',  ( 8.749999999999918288, 12.50000000000000000, 7.188010851410848723 ) ) ;
#11763=DIRECTION ( 'NONE',  ( 0.000000000000000000, 0.000000000000000000, -1.000000000000000000 ) ) ;
#11764=VECTOR ( 'NONE', #53236, 1000.000000000000000 ) ;
#11765=CONICAL_SURFACE ( 'NONE', #95404, 0.1000000000000002554, 0.003490658503988666988 ) ;
#11766=EDGE_LOOP ( 'NONE', ( #60812, #85043 ) ) ;
#11767=CIRCLE ( 'NONE', #20190, 0.06509327318403745899 ) ;
#11768=CARTESIAN_POINT ( 'NONE',  ( 5.849999999999931255, 2.500000000000000000, 2.757883832488649656 ) ) ;
#11769=FACE_OUTER_BOUND ( 'NONE', #57869, .T. ) ;
#11770=DIRECTION ( 'NONE',  ( 0.000000000000000000, 0.000000000000000000, 1.000000000000000000 ) ) ;
#11771=ORIENTED_EDGE ( 'NONE', *, *, #119343, .F. ) ;
#11772=VERTEX_POINT ( 'NONE', #80753 ) ;
#11773=DIRECTION ( 'NONE',  ( 0.000000000000000000, -0.000000000000000000, 1.000000000000000000 ) ) ;
#11774=ORIENTED_EDGE ( 'NONE', *, *, #39714, .T. ) ;
#11775=FACE_OUTER_BOUND ( 'NONE', #95722, .T. ) ;
#11776=CARTESIAN_POINT ( 'NONE',  ( -0.8500000000000390576, 2.500000000000000000, -6.595190528383302109 ) ) ;
#11777=ADVANCED_FACE ( 'NONE', ( #42110 ), #121959, .T. ) ;
#11778=DIRECTION ( 'NONE',  ( -0.000000000000000000, 1.000000000000000000, -0.000000000000000000 ) ) ;
#11779=EDGE_LOOP ( 'NONE', ( #68961, #44780 ) ) ;
#11780=CARTESIAN_POINT ( 'NONE',  ( -3.350000000000028955, 2.500000000000000000, 7.188010851410848723 ) ) ;
#11781=ADVANCED_FACE ( 'NONE', ( #32954 ), #70925, .T. ) ;
#11782=DIRECTION ( 'NONE',  ( -0.000000000000000000, -1.000000000000000000, -0.000000000000000000 ) ) ;
#11784=CARTESIAN_POINT ( 'NONE',  ( -12.89999999999999147, 2.500000000000000000, 3.737306695894644371 ) ) ;
#11785=CARTESIAN_POINT ( 'NONE',  ( 1.249999999999952038, 2.500000000000000000, 2.857883832488649301 ) ) ;
#11786=AXIS2_PLACEMENT_3D ( 'NONE', #122876, #91469, #1786 ) ;
#11787=CARTESIAN_POINT ( 'NONE',  ( 15.19999999999989271, 2.500000000000000000, -0.3464101615137783474 ) ) ;
#11788=EDGE_CURVE ( 'NONE', #79738, #31609, #112142, .T. ) ;
#11789=ORIENTED_EDGE ( 'NONE', *, *, #39111, .T. ) ;
#11790=ORIENTED_EDGE ( 'NONE', *, *, #86360, .F. ) ;
#11791=DIRECTION ( 'NONE',  ( 0.000000000000000000, 1.000000000000000000, 0.000000000000000000 ) ) ;
#11792=ORIENTED_EDGE ( 'NONE', *, *, #42174, .F. ) ;
#11793=AXIS2_PLACEMENT_3D ( 'NONE', #98481, #88681, #79514 ) ;
#11794=AXIS2_PLACEMENT_3D ( 'NONE', #125957, #7473, #116780 ) ;
#11795=CARTESIAN_POINT ( 'NONE',  ( -3.750000000000029310, 2.500000000000000000, -7.088010851410853519 ) ) ;
#11796=EDGE_LOOP ( 'NONE', ( #104407, #26612 ) ) ;
#11797=ORIENTED_EDGE ( 'NONE', *, *, #65518, .F. ) ;
#11798=ORIENTED_EDGE ( 'NONE', *, *, #8272, .T. ) ;
#11799=CARTESIAN_POINT ( 'NONE',  ( -15.39999999999998082, 2.500000000000000000, 0.5928203230275517210 ) ) ;
#11800=CIRCLE ( 'NONE', #34809, 0.06509327318403745899 ) ;
#11801=FACE_OUTER_BOUND ( 'NONE', #35238, .T. ) ;
#11802=CARTESIAN_POINT ( 'NONE',  ( -3.150000000000029221, 2.500000000000000000, 2.511473670974873507 ) ) ;
#11804=CARTESIAN_POINT ( 'NONE',  ( -12.04999999999999538, 2.500000000000000000, 2.065063509461097624 ) ) ;
#11805=DIRECTION ( 'NONE',  ( -0.000000000000000000, -1.000000000000000000, -0.000000000000000000 ) ) ;
#11806=CARTESIAN_POINT ( 'NONE',  ( -10.60000000000000142, 2.500000000000000000, 3.883716857408421319 ) ) ;
#11807=DIRECTION ( 'NONE',  ( 0.000000000000000000, 0.000000000000000000, -1.000000000000000000 ) ) ;
#11808=CARTESIAN_POINT ( 'NONE',  ( -8.750000000000007105, 2.500000000000000000, 7.288010851410849256 ) ) ;
#11809=FACE_OUTER_BOUND ( 'NONE', #50382, .T. ) ;
#11810=CONICAL_SURFACE ( 'NONE', #55725, 0.09999999999999982514, 0.003490658503988666988 ) ;
#11811=ORIENTED_EDGE ( 'NONE', *, *, #64171, .F. ) ;
#11812=CONICAL_SURFACE ( 'NONE', #95446, 0.09999999999999982514, 0.003490658503988666988 ) ;
#11813=AXIS2_PLACEMENT_3D ( 'NONE', #123650, #101459, #71333 ) ;
#11814=CARTESIAN_POINT ( 'NONE',  ( 12.29999999999990656, 2.500000000000000000, 3.983716857408420964 ) ) ;
#11815=VERTEX_POINT ( 'NONE', #102322 ) ;
#11816=ORIENTED_EDGE ( 'NONE', *, *, #4207, .F. ) ;
#11817=FACE_OUTER_BOUND ( 'NONE', #42637, .T. ) ;
#11819=DIRECTION ( 'NONE',  ( -0.000000000000000000, 1.000000000000000000, -0.000000000000000000 ) ) ;
#11820=ADVANCED_FACE ( 'NONE', ( #100384 ), #128378, .T. ) ;
#11821=CARTESIAN_POINT ( 'NONE',  ( 11.24999999999991118, 2.500000000000000000, -2.857883832488653741 ) ) ;
#11822=CARTESIAN_POINT ( 'NONE',  ( -11.05000000000000071, 12.50000000000000000, 2.511473670974873507 ) ) ;
#11823=FACE_OUTER_BOUND ( 'NONE', #53396, .T. ) ;
#11824=DIRECTION ( 'NONE',  ( 0.000000000000000000, 1.000000000000000000, 0.000000000000000000 ) ) ;
#11825=ORIENTED_EDGE ( 'NONE', *, *, #96079, .T. ) ;
#11826=EDGE_LOOP ( 'NONE', ( #126598, #96316 ) ) ;
#11827=ORIENTED_EDGE ( 'NONE', *, *, #52198, .F. ) ;
#11828=VERTEX_POINT ( 'NONE', #70285 ) ;
#11829=EDGE_CURVE ( 'NONE', #61230, #14447, #117874, .T. ) ;
#11830=EDGE_CURVE ( 'NONE', #116790, #111264, #21167, .T. ) ;
#11831=EDGE_LOOP ( 'NONE', ( #9628, #70937, #65606, #50521 ) ) ;
#11832=DIRECTION ( 'NONE',  ( 0.000000000000000000, 0.000000000000000000, -1.000000000000000000 ) ) ;
#11833=CARTESIAN_POINT ( 'NONE',  ( 0.1999999999999627909, 2.500000000000000000, 0.2464101615137758439 ) ) ;
#11834=AXIS2_PLACEMENT_3D ( 'NONE', #32098, #31446, #121101 ) ;
#11836=CONICAL_SURFACE ( 'NONE', #66126, 0.1000000000000002554, 0.003490658503988666988 ) ;
#11837=DIRECTION ( 'NONE',  ( 0.000000000000000000, 1.000000000000000000, 0.000000000000000000 ) ) ;
#11838=DIRECTION ( 'NONE',  ( 0.000000000000000000, -0.9999939076577903929, 0.003490651415223739937 ) ) ;
#11839=ORIENTED_EDGE ( 'NONE', *, *, #102423, .T. ) ;
#11840=DIRECTION ( 'NONE',  ( 0.000000000000000000, 0.000000000000000000, -1.000000000000000000 ) ) ;
#11841=DIRECTION ( 'NONE',  ( -0.000000000000000000, -1.000000000000000000, -0.000000000000000000 ) ) ;
#11842=EDGE_CURVE ( 'NONE', #55864, #47422, #52563, .T. ) ;
#11843=CARTESIAN_POINT ( 'NONE',  ( -8.350000000000012079, 2.500000000000000000, 1.372243186433545370 ) ) ;
#11844=DIRECTION ( 'NONE',  ( 0.000000000000000000, 1.000000000000000000, 0.000000000000000000 ) ) ;
#11845=AXIS2_PLACEMENT_3D ( 'NONE', #59712, #756, #129099 ) ;
#11846=AXIS2_PLACEMENT_3D ( 'NONE', #35117, #75025, #65175 ) ;
#11848=VERTEX_POINT ( 'NONE', #91855 ) ;
#11849=ORIENTED_EDGE ( 'NONE', *, *, #63749, .T. ) ;
#11850=ORIENTED_EDGE ( 'NONE', *, *, #56555, .T. ) ;
#11851=DIRECTION ( 'NONE',  ( 0.000000000000000000, -0.9999939076577903929, 0.003490651415223739937 ) ) ;
#11852=VERTEX_POINT ( 'NONE', #81401 ) ;
#11853=AXIS2_PLACEMENT_3D ( 'NONE', #102172, #34742, #41967 ) ;
#11854=VECTOR ( 'NONE', #87714, 1000.000000000000000 ) ;
#11855=DIRECTION ( 'NONE',  ( 0.000000000000000000, 0.000000000000000000, -1.000000000000000000 ) ) ;
#11856=FACE_OUTER_BOUND ( 'NONE', #92836, .T. ) ;
#11857=AXIS2_PLACEMENT_3D ( 'NONE', #80192, #102408, #91939 ) ;
#11858=EDGE_LOOP ( 'NONE', ( #96103, #6259 ) ) ;
#11859=DIRECTION ( 'NONE',  ( -4.274815082592931898E-19, -0.9999939076577903929, -0.003490651415223739937 ) ) ;
#11860=CARTESIAN_POINT ( 'NONE',  ( -10.80000000000000249, 2.500000000000000000, -4.330127018922197202 ) ) ;
#11861=CARTESIAN_POINT ( 'NONE',  ( 6.849999999999929479, 12.50000000000000000, 6.213873640053558134 ) ) ;
#11862=DIRECTION ( 'NONE',  ( 0.000000000000000000, 1.000000000000000000, 0.000000000000000000 ) ) ;
#11863=ADVANCED_FACE ( 'NONE', ( #82691 ), #38493, .T. ) ;
#11864=CARTESIAN_POINT ( 'NONE',  ( -5.850000000000021849, 2.500000000000000000, -1.472243186433550122 ) ) ;
#11865=ORIENTED_EDGE ( 'NONE', *, *, #84264, .T. ) ;
#11866=EDGE_LOOP ( 'NONE', ( #71046, #65402 ) ) ;
#11867=ADVANCED_FACE ( 'NONE', ( #42780 ), #57252, .T. ) ;
#11868=CARTESIAN_POINT ( 'NONE',  ( -7.700000000000016165, 12.50000000000000000, -4.048810130592463530 ) ) ;
#11869=AXIS2_PLACEMENT_3D ( 'NONE', #15476, #96606, #94687 ) ;
#11870=DIRECTION ( 'NONE',  ( 0.000000000000000000, -0.000000000000000000, 1.000000000000000000 ) ) ;
#11871=CIRCLE ( 'NONE', #127112, 0.1000000000000000472 ) ;
#11872=ADVANCED_FACE ( 'NONE', ( #120669 ), #4999, .T. ) ;
#11873=DIRECTION ( 'NONE',  ( -0.000000000000000000, 1.000000000000000000, -0.000000000000000000 ) ) ;
#11874=CIRCLE ( 'NONE', #60224, 0.06509327318403745899 ) ;
#11875=DIRECTION ( 'NONE',  ( -4.274815082592931898E-19, -0.9999939076577903929, -0.003490651415223739937 ) ) ;
#11876=ORIENTED_EDGE ( 'NONE', *, *, #21955, .F. ) ;
#11877=VECTOR ( 'NONE', #89810, 1000.000000000000000 ) ;
#11878=EDGE_CURVE ( 'NONE', #78632, #122009, #99013, .T. ) ;
#11879=EDGE_CURVE ( 'NONE', #68006, #3892, #111483, .T. ) ;
#11880=ORIENTED_EDGE ( 'NONE', *, *, #45133, .T. ) ;
#11881=CARTESIAN_POINT ( 'NONE',  ( -1.650000000000034328, 2.500000000000000000, -2.857883832488653741 ) ) ;
#11882=PLANE ( 'NONE',  #124106 ) ;
#11883=EDGE_CURVE ( 'NONE', #68389, #124065, #111632, .T. ) ;
#11884=VECTOR ( 'NONE', #16091, 1000.000000000000000 ) ;
#11885=DIRECTION ( 'NONE',  ( 0.000000000000000000, -0.9999939076577903929, 0.003490651415223739937 ) ) ;
#11886=AXIS2_PLACEMENT_3D ( 'NONE', #99357, #9675, #78441 ) ;
#11887=DIRECTION ( 'NONE',  ( -0.000000000000000000, -1.000000000000000000, -0.000000000000000000 ) ) ;
#11888=VERTEX_POINT ( 'NONE', #58946 ) ;
#11889=DIRECTION ( 'NONE',  ( 0.000000000000000000, 0.000000000000000000, -1.000000000000000000 ) ) ;
#11890=AXIS2_PLACEMENT_3D ( 'NONE', #49885, #119896, #81264 ) ;
#11891=ADVANCED_FACE ( 'NONE', ( #49139 ), #126204, .T. ) ;
#11892=LINE ( 'NONE', #52459, #59920 ) ;
#11893=VERTEX_POINT ( 'NONE', #47843 ) ;
#11894=CARTESIAN_POINT ( 'NONE',  ( -5.850000000000021849, 12.50000000000000000, -5.737276932171712751 ) ) ;
#11895=CIRCLE ( 'NONE', #43232, 0.06509327318403745899 ) ;
#11896=EDGE_LOOP ( 'NONE', ( #115960, #32524, #128395, #93765 ) ) ;
#11897=EDGE_CURVE ( 'NONE', #102161, #7340, #87736, .T. ) ;
#11898=DIRECTION ( 'NONE',  ( 0.000000000000000000, 0.000000000000000000, 1.000000000000000000 ) ) ;
#11899=EDGE_LOOP ( 'NONE', ( #12782, #25185, #58671, #109468 ) ) ;
#11900=AXIS2_PLACEMENT_3D ( 'NONE', #117547, #47562, #87459 ) ;
#11901=AXIS2_PLACEMENT_3D ( 'NONE', #26762, #125588, #75846 ) ;
#11902=EDGE_LOOP ( 'NONE', ( #62032, #17411 ) ) ;
#11903=CARTESIAN_POINT ( 'NONE',  ( -3.350000000000028955, 2.500000000000000000, 2.065063509461097624 ) ) ;
#11904=DIRECTION ( 'NONE',  ( -0.000000000000000000, 1.000000000000000000, -0.000000000000000000 ) ) ;
#11905=ORIENTED_EDGE ( 'NONE', *, *, #110981, .T. ) ;
#11906=VERTEX_POINT ( 'NONE', #8525 ) ;
#11907=DIRECTION ( 'NONE',  ( 0.000000000000000000, 0.000000000000000000, 1.000000000000000000 ) ) ;
#11908=DIRECTION ( 'NONE',  ( -0.000000000000000000, 1.000000000000000000, -0.000000000000000000 ) ) ;
#11911=DIRECTION ( 'NONE',  ( 0.000000000000000000, 0.000000000000000000, 1.000000000000000000 ) ) ;
#11912=CARTESIAN_POINT ( 'NONE',  ( -9.400000000000009237, 2.500000000000000000, -4.676537180435974328 ) ) ;
#11913=LINE ( 'NONE', #72778, #115699 ) ;
#11914=DIRECTION ( 'NONE',  ( 0.000000000000000000, 1.000000000000000000, 0.000000000000000000 ) ) ;
#11915=DIRECTION ( 'NONE',  ( 0.000000000000000000, -0.000000000000000000, 1.000000000000000000 ) ) ;
#11916=VECTOR ( 'NONE', #47542, 1000.000000000000000 ) ;
#11917=ORIENTED_EDGE ( 'NONE', *, *, #4292, .F. ) ;
#11918=ORIENTED_EDGE ( 'NONE', *, *, #93928, .F. ) ;
#11919=DIRECTION ( 'NONE',  ( 0.000000000000000000, 0.000000000000000000, 1.000000000000000000 ) ) ;
#11920=ORIENTED_EDGE ( 'NONE', *, *, #112984, .T. ) ;
#11921=DIRECTION ( 'NONE',  ( 0.000000000000000000, 0.000000000000000000, -1.000000000000000000 ) ) ;
#11922=CARTESIAN_POINT ( 'NONE',  ( -5.600000000000020073, 2.500000000000000000, 4.676537180435972552 ) ) ;
#11923=DIRECTION ( 'NONE',  ( 0.000000000000000000, -0.9999939076577903929, 0.003490651415223739937 ) ) ;
#11924=ORIENTED_EDGE ( 'NONE', *, *, #9965, .F. ) ;
#11925=ORIENTED_EDGE ( 'NONE', *, *, #129080, .F. ) ;
#11926=FACE_BOUND ( 'NONE', #37732, .T. ) ;
#11927=VERTEX_POINT ( 'NONE', #88372 ) ;
#11928=FACE_OUTER_BOUND ( 'NONE', #84453, .T. ) ;
#11929=CARTESIAN_POINT ( 'NONE',  ( -13.34999999999999076, 2.500000000000000000, 1.372243186433549367 ) ) ;
#11930=CARTESIAN_POINT ( 'NONE',  ( 3.949999999999942446, 2.500000000000000000, -6.841600689897078702 ) ) ;
#11931=DIRECTION ( 'NONE',  ( 0.000000000000000000, 1.000000000000000000, 0.000000000000000000 ) ) ;
#11932=CONICAL_SURFACE ( 'NONE', #43352, 0.09999999999999999167, 0.003490658503988666988 ) ;
#11933=EDGE_CURVE ( 'NONE', #117447, #56076, #127670, .T. ) ;
#11934=DIRECTION ( 'NONE',  ( -4.274815082592931898E-19, -0.9999939076577903929, -0.003490651415223739937 ) ) ;
#11935=CIRCLE ( 'NONE', #91356, 0.06509327318403745899 ) ;
#11936=DIRECTION ( 'NONE',  ( 0.000000000000000000, 0.000000000000000000, 1.000000000000000000 ) ) ;
#11937=FACE_OUTER_BOUND ( 'NONE', #70291, .T. ) ;
#11939=FACE_OUTER_BOUND ( 'NONE', #125683, .T. ) ;
#11940=DIRECTION ( 'NONE',  ( 0.000000000000000000, 0.000000000000000000, -1.000000000000000000 ) ) ;
#11941=DIRECTION ( 'NONE',  ( 0.000000000000000000, 0.000000000000000000, -1.000000000000000000 ) ) ;
#11942=AXIS2_PLACEMENT_3D ( 'NONE', #117133, #89638, #129587 ) ;
#11943=CIRCLE ( 'NONE', #53711, 0.06509327318403741736 ) ;
#11944=EDGE_CURVE ( 'NONE', #108909, #122396, #46795, .T. ) ;
#11945=ORIENTED_EDGE ( 'NONE', *, *, #116953, .T. ) ;
#11946=EDGE_LOOP ( 'NONE', ( #28845, #109274 ) ) ;
#11947=VERTEX_POINT ( 'NONE', #79865 ) ;
#11948=DIRECTION ( 'NONE',  ( 0.000000000000000000, 0.000000000000000000, 1.000000000000000000 ) ) ;
#11949=EDGE_LOOP ( 'NONE', ( #63197, #90478, #103, #83746 ) ) ;
#11950=CARTESIAN_POINT ( 'NONE',  ( -3.550000000000027356, 2.500000000000000000, 1.718653347947321386 ) ) ;
#11951=FACE_OUTER_BOUND ( 'NONE', #76478, .T. ) ;
#11952=ORIENTED_EDGE ( 'NONE', *, *, #48469, .F. ) ;
#11953=ORIENTED_EDGE ( 'NONE', *, *, #96476, .F. ) ;
#11954=VERTEX_POINT ( 'NONE', #58310 ) ;
#11955=FACE_OUTER_BOUND ( 'NONE', #11033, .T. ) ;
#11957=AXIS2_PLACEMENT_3D ( 'NONE', #122360, #51047, #90956 ) ;
#11958=DIRECTION ( 'NONE',  ( 0.000000000000000000, -0.000000000000000000, 1.000000000000000000 ) ) ;
#11959=DIRECTION ( 'NONE',  ( -0.000000000000000000, -1.000000000000000000, -0.000000000000000000 ) ) ;
#11960=CARTESIAN_POINT ( 'NONE',  ( -11.24999999999996447, 2.500000000000000000, -2.065063509461098068 ) ) ;
#11961=DIRECTION ( 'NONE',  ( 0.000000000000000000, -0.9999939076577903929, 0.003490651415223739937 ) ) ;
#11962=DIRECTION ( 'NONE',  ( 0.000000000000000000, 0.000000000000000000, -1.000000000000000000 ) ) ;
#11963=VERTEX_POINT ( 'NONE', #68100 ) ;
#11964=DIRECTION ( 'NONE',  ( 0.000000000000000000, 0.000000000000000000, -1.000000000000000000 ) ) ;
#11965=EDGE_LOOP ( 'NONE', ( #85121, #33684, #95495, #121589 ) ) ;
#11966=VERTEX_POINT ( 'NONE', #109976 ) ;
#11967=VERTEX_POINT ( 'NONE', #99520 ) ;
#11969=EDGE_LOOP ( 'NONE', ( #108849, #122761, #40969, #31708 ) ) ;
#11970=ORIENTED_EDGE ( 'NONE', *, *, #23707, .T. ) ;
#11971=ORIENTED_EDGE ( 'NONE', *, *, #62139, .F. ) ;
#11972=CONICAL_SURFACE ( 'NONE', #85125, 0.1000000000000002554, 0.003490658503988666988 ) ;
#11973=AXIS2_PLACEMENT_3D ( 'NONE', #117201, #27543, #108055 ) ;
#11974=DIRECTION ( 'NONE',  ( 0.000000000000000000, 0.000000000000000000, -1.000000000000000000 ) ) ;
#11975=EDGE_CURVE ( 'NONE', #59442, #12555, #128997, .T. ) ;
#11977=DIRECTION ( 'NONE',  ( -0.000000000000000000, 1.000000000000000000, -0.000000000000000000 ) ) ;
#11978=AXIS2_PLACEMENT_3D ( 'NONE', #6848, #84791, #24582 ) ;
#11979=CARTESIAN_POINT ( 'NONE',  ( 7.049999999999928768, 2.500000000000000000, 6.495190528383297135 ) ) ;
#11980=DIRECTION ( 'NONE',  ( 0.000000000000000000, 0.000000000000000000, 1.000000000000000000 ) ) ;
#11981=DIRECTION ( 'NONE',  ( 0.000000000000000000, 0.000000000000000000, 1.000000000000000000 ) ) ;
#11982=CIRCLE ( 'NONE', #122799, 0.06509327318403745899 ) ;
#11983=DIRECTION ( 'NONE',  ( 0.000000000000000000, 0.000000000000000000, 1.000000000000000000 ) ) ;
#11984=AXIS2_PLACEMENT_3D ( 'NONE', #1772, #2405, #23341 ) ;
#11985=ADVANCED_FACE ( 'NONE', ( #89045 ), #128343, .T. ) ;
#11986=EDGE_LOOP ( 'NONE', ( #22574, #100256, #80191, #62413 ) ) ;
#11987=AXIS2_PLACEMENT_3D ( 'NONE', #115156, #63524, #94256 ) ;
#11988=CIRCLE ( 'NONE', #22485, 0.1000000000000002554 ) ;
#11989=DIRECTION ( 'NONE',  ( 0.000000000000000000, 0.000000000000000000, -1.000000000000000000 ) ) ;
#11991=DIRECTION ( 'NONE',  ( -0.000000000000000000, -1.000000000000000000, -0.000000000000000000 ) ) ;
#11992=VERTEX_POINT ( 'NONE', #69392 ) ;
#11993=DIRECTION ( 'NONE',  ( -4.274815082592931898E-19, -0.9999939076577903929, -0.003490651415223739937 ) ) ;
#11994=ADVANCED_FACE ( 'NONE', ( #49782 ), #15464, .T. ) ;
#11995=CONICAL_SURFACE ( 'NONE', #78918, 0.09999999999999982514, 0.003490658503988666988 ) ;
#11996=EDGE_CURVE ( 'NONE', #15907, #78758, #98207, .T. ) ;
#11998=LINE ( 'NONE', #53865, #15059 ) ;
#11999=ADVANCED_FACE ( 'NONE', ( #30140 ), #70051, .T. ) ;
#12000=CARTESIAN_POINT ( 'NONE',  ( -11.24999999999999822, 2.500000000000000000, 1.372243186433545370 ) ) ;
#12001=ORIENTED_EDGE ( 'NONE', *, *, #76302, .F. ) ;
#12002=ORIENTED_EDGE ( 'NONE', *, *, #66404, .T. ) ;
#12003=CARTESIAN_POINT ( 'NONE',  ( 2.499999999999945377, 12.50000000000000000, 4.957854068765711553 ) ) ;
#12004=DIRECTION ( 'NONE',  ( 0.000000000000000000, 0.000000000000000000, 1.000000000000000000 ) ) ;
#12006=DIRECTION ( 'NONE',  ( 0.000000000000000000, 0.000000000000000000, 1.000000000000000000 ) ) ;
#12007=FACE_OUTER_BOUND ( 'NONE', #111756, .T. ) ;
#12008=DIRECTION ( 'NONE',  ( -0.000000000000000000, -1.000000000000000000, -0.000000000000000000 ) ) ;
#12009=ORIENTED_EDGE ( 'NONE', *, *, #1542, .F. ) ;
#12010=DIRECTION ( 'NONE',  ( -0.000000000000000000, 1.000000000000000000, -0.000000000000000000 ) ) ;
#12011=CONICAL_SURFACE ( 'NONE', #72668, 0.1000000000000000472, 0.003490658503988666988 ) ;
#12012=EDGE_LOOP ( 'NONE', ( #70755, #58312 ) ) ;
#12013=DIRECTION ( 'NONE',  ( 0.000000000000000000, 1.000000000000000000, 0.000000000000000000 ) ) ;
#12014=DIRECTION ( 'NONE',  ( 0.000000000000000000, 1.000000000000000000, 0.000000000000000000 ) ) ;
#12015=DIRECTION ( 'NONE',  ( -0.000000000000000000, -1.000000000000000000, -0.000000000000000000 ) ) ;
#12016=DIRECTION ( 'NONE',  ( 0.000000000000000000, 1.000000000000000000, 0.000000000000000000 ) ) ;
#12017=DIRECTION ( 'NONE',  ( -0.000000000000000000, -1.000000000000000000, -0.000000000000000000 ) ) ;
#12018=DIRECTION ( 'NONE',  ( -0.000000000000000000, -1.000000000000000000, -0.000000000000000000 ) ) ;
#12019=ORIENTED_EDGE ( 'NONE', *, *, #20201, .F. ) ;
#12020=CIRCLE ( 'NONE', #24647, 0.06509327318403745899 ) ;
#12021=CARTESIAN_POINT ( 'NONE',  ( -7.300000000000018474, 12.50000000000000000, 0.2813168883297361700 ) ) ;
#12022=ADVANCED_FACE ( 'NONE', ( #100159 ), #115728, .T. ) ;
#12023=VECTOR ( 'NONE', #24427, 1000.000000000000000 ) ;
#12024=CARTESIAN_POINT ( 'NONE',  ( 1.049999999999954525, 12.50000000000000000, -2.576566944158915184 ) ) ;
#12025=DIRECTION ( 'NONE',  ( 0.000000000000000000, 1.000000000000000000, 0.000000000000000000 ) ) ;
#12026=ORIENTED_EDGE ( 'NONE', *, *, #92064, .T. ) ;
#12027=ORIENTED_EDGE ( 'NONE', *, *, #34644, .F. ) ;
#12028=CIRCLE ( 'NONE', #28779, 0.09999999999999982514 ) ;
#12029=ADVANCED_FACE ( 'NONE', ( #30786 ), #30078, .T. ) ;
#12030=CARTESIAN_POINT ( 'NONE',  ( -10.65000000000000391, 12.50000000000000000, -1.883746621131359600 ) ) ;
#12031=AXIS2_PLACEMENT_3D ( 'NONE', #85847, #126445, #104843 ) ;
#12032=ORIENTED_EDGE ( 'NONE', *, *, #92905, .T. ) ;
#12033=EDGE_LOOP ( 'NONE', ( #66861, #5052, #33704, #126099 ) ) ;
#12034=CARTESIAN_POINT ( 'NONE',  ( 11.44999999999990870, 2.500000000000000000, 6.841600689897072485 ) ) ;
#12035=ADVANCED_FACE ( 'NONE', ( #90309 ), #80526, .T. ) ;
#12036=EDGE_LOOP ( 'NONE', ( #19805, #64911, #84298, #48166 ) ) ;
#12037=CARTESIAN_POINT ( 'NONE',  ( 0.8499999999999553468, 2.500000000000000000, -2.857883832488653741 ) ) ;
#12038=DIRECTION ( 'NONE',  ( -0.000000000000000000, 1.000000000000000000, -0.000000000000000000 ) ) ;
#12039=EDGE_CURVE ( 'NONE', #89331, #55129, #122004, .T. ) ;
#12040=CARTESIAN_POINT ( 'NONE',  ( 16.72050902516894411, 2.552201582241256705, 5.918448581777647988 ) ) ;
#12041=CONICAL_SURFACE ( 'NONE', #63998, 0.1000000000000000472, 0.003490658503988666988 ) ;
#12042=EDGE_CURVE ( 'NONE', #72591, #47419, #23805, .T. ) ;
#12043=ORIENTED_EDGE ( 'NONE', *, *, #71907, .T. ) ;
#12044=CIRCLE ( 'NONE', #129061, 0.06509327318403745899 ) ;
#12045=DIRECTION ( 'NONE',  ( 0.000000000000000000, -0.000000000000000000, 1.000000000000000000 ) ) ;
#12046=EDGE_CURVE ( 'NONE', #100514, #11992, #34282, .T. ) ;
#12047=DIRECTION ( 'NONE',  ( 0.000000000000000000, 1.000000000000000000, 0.000000000000000000 ) ) ;
#12048=AXIS2_PLACEMENT_3D ( 'NONE', #10844, #91364, #33734 ) ;
#12049=EDGE_LOOP ( 'NONE', ( #89291, #69615 ) ) ;
#12050=ADVANCED_FACE ( 'NONE', ( #113180 ), #107422, .T. ) ;
#12051=VECTOR ( 'NONE', #10777, 1000.000000000000000 ) ;
#12052=EDGE_CURVE ( 'NONE', #27361, #51042, #51006, .T. ) ;
#12053=ORIENTED_EDGE ( 'NONE', *, *, #23131, .F. ) ;
#12054=EDGE_LOOP ( 'NONE', ( #67971, #85457, #48828, #3473 ) ) ;
#12055=DIRECTION ( 'NONE',  ( 0.000000000000000000, 0.000000000000000000, 1.000000000000000000 ) ) ;
#12056=DIRECTION ( 'NONE',  ( 0.000000000000000000, -0.9999939076577903929, 0.003490651415223739937 ) ) ;
#12057=DIRECTION ( 'NONE',  ( -0.000000000000000000, -1.000000000000000000, -0.000000000000000000 ) ) ;
#12058=FACE_BOUND ( 'NONE', #55141, .T. ) ;
#12059=EDGE_LOOP ( 'NONE', ( #94720, #80895 ) ) ;
#12060=VECTOR ( 'NONE', #81657, 1000.000000000000000 ) ;
#12061=DIRECTION ( 'NONE',  ( 0.000000000000000000, 0.000000000000000000, 1.000000000000000000 ) ) ;
#12062=FACE_OUTER_BOUND ( 'NONE', #50018, .T. ) ;
#12063=VECTOR ( 'NONE', #8335, 1000.000000000000000 ) ;
#12064=ORIENTED_EDGE ( 'NONE', *, *, #2256, .T. ) ;
#12065=DIRECTION ( 'NONE',  ( 0.000000000000000000, 0.000000000000000000, -1.000000000000000000 ) ) ;
#12066=DIRECTION ( 'NONE',  ( -0.000000000000000000, -1.000000000000000000, -0.000000000000000000 ) ) ;
#12067=CONICAL_SURFACE ( 'NONE', #127107, 0.09999999999999982514, 0.003490658503988666988 ) ;
#12068=CARTESIAN_POINT ( 'NONE',  ( -14.39999999999998614, 2.500000000000000000, -0.4464101615137760493 ) ) ;
#12069=CARTESIAN_POINT ( 'NONE',  ( -3.350000000000032507, 12.50000000000000000, -6.495190528383302464 ) ) ;
#12070=FACE_OUTER_BOUND ( 'NONE', #60476, .T. ) ;
#12071=CARTESIAN_POINT ( 'NONE',  ( 8.949999999999919353, 2.500000000000000000, 2.611473670974873151 ) ) ;
#12072=AXIS2_PLACEMENT_3D ( 'NONE', #55253, #46714, #27705 ) ;
#12073=DIRECTION ( 'NONE',  ( -4.274815082592931898E-19, -0.9999939076577903929, -0.003490651415223739937 ) ) ;
#12074=CONICAL_SURFACE ( 'NONE', #89445, 0.1000000000000002554, 0.003490658503988666988 ) ;
#12075=CONICAL_SURFACE ( 'NONE', #116628, 0.1000000000000000472, 0.003490658503988666988 ) ;
#12076=ORIENTED_EDGE ( 'NONE', *, *, #9630, .F. ) ;
#12077=VERTEX_POINT ( 'NONE', #51070 ) ;
#12078=ORIENTED_EDGE ( 'NONE', *, *, #86, .T. ) ;
#12079=ORIENTED_EDGE ( 'NONE', *, *, #56090, .T. ) ;
#12080=CARTESIAN_POINT ( 'NONE',  ( -3.150000000000029221, 2.500000000000000000, -1.918653347947326004 ) ) ;
#12081=CARTESIAN_POINT ( 'NONE',  ( -5.400000000000024336, 12.50000000000000000, -3.637306695894650055 ) ) ;
#12082=CONICAL_SURFACE ( 'NONE', #20512, 0.1000000000000000472, 0.003490658503988666988 ) ;
#12083=ORIENTED_EDGE ( 'NONE', *, *, #51055, .T. ) ;
#12084=FACE_BOUND ( 'NONE', #51681, .T. ) ;
#12085=DIRECTION ( 'NONE',  ( 0.000000000000000000, 1.000000000000000000, 0.000000000000000000 ) ) ;
#12086=CARTESIAN_POINT ( 'NONE',  ( -3.100000000000028955, 2.500000000000000000, 4.083716857408421497 ) ) ;
#12087=DIRECTION ( 'NONE',  ( -4.274815082592931898E-19, -0.9999939076577903929, -0.003490651415223739937 ) ) ;
#12088=CIRCLE ( 'NONE', #93572, 0.1000000000000002554 ) ;
#12089=VECTOR ( 'NONE', #127788, 1000.000000000000000 ) ;
#12090=DIRECTION ( 'NONE',  ( 0.000000000000000000, 1.000000000000000000, 0.000000000000000000 ) ) ;
#12091=DIRECTION ( 'NONE',  ( 0.000000000000000000, 1.000000000000000000, 0.000000000000000000 ) ) ;
#12092=DIRECTION ( 'NONE',  ( 0.000000000000000000, 0.000000000000000000, 1.000000000000000000 ) ) ;
#12093=LINE ( 'NONE', #102419, #78887 ) ;
#12094=CARTESIAN_POINT ( 'NONE',  ( -9.400000000000007461, 12.50000000000000000, 0.2813168883297361700 ) ) ;
#12095=PLANE ( 'NONE',  #68507 ) ;
#12096=ORIENTED_EDGE ( 'NONE', *, *, #44391, .T. ) ;
#12097=VERTEX_POINT ( 'NONE', #61531 ) ;
#12098=EDGE_CURVE ( 'NONE', #46427, #4150, #55196, .T. ) ;
#12099=ORIENTED_EDGE ( 'NONE', *, *, #94787, .T. ) ;
#12100=VERTEX_POINT ( 'NONE', #43833 ) ;
#12101=VERTEX_POINT ( 'NONE', #13689 ) ;
#12102=EDGE_LOOP ( 'NONE', ( #80291, #14379 ) ) ;
#12103=EDGE_LOOP ( 'NONE', ( #81593, #41132 ) ) ;
#12104=CARTESIAN_POINT ( 'NONE',  ( 1.449999999999950440, 2.500000000000000000, 6.248780366869520542 ) ) ;
#12105=ORIENTED_EDGE ( 'NONE', *, *, #53001, .F. ) ;
#12106=ORIENTED_EDGE ( 'NONE', *, *, #47238, .F. ) ;
#12107=CARTESIAN_POINT ( 'NONE',  ( -5.650000000000023448, 12.50000000000000000, -6.906693963081115939 ) ) ;
#12108=DIRECTION ( 'NONE',  ( 0.000000000000000000, -0.000000000000000000, 1.000000000000000000 ) ) ;
#12109=CARTESIAN_POINT ( 'NONE',  ( -11.04999999999999893, 2.500000000000000000, 6.148780366869520009 ) ) ;
#12110=DIRECTION ( 'NONE',  ( -0.000000000000000000, 1.000000000000000000, -0.000000000000000000 ) ) ;
#12111=AXIS2_PLACEMENT_3D ( 'NONE', #69900, #9684, #127528 ) ;
#12112=ORIENTED_EDGE ( 'NONE', *, *, #31675, .T. ) ;
#12113=CARTESIAN_POINT ( 'NONE',  ( 5.399999999999934630, 12.50000000000000000, -0.7579135962115917113 ) ) ;
#12114=AXIS2_PLACEMENT_3D ( 'NONE', #32288, #110181, #40813 ) ;
#12115=ORIENTED_EDGE ( 'NONE', *, *, #98332, .T. ) ;
#12116=AXIS2_PLACEMENT_3D ( 'NONE', #109435, #39434, #107501 ) ;
#12117=ORIENTED_EDGE ( 'NONE', *, *, #7478, .F. ) ;
#12119=DIRECTION ( 'NONE',  ( 0.000000000000000000, 1.000000000000000000, 0.000000000000000000 ) ) ;
#12120=EDGE_LOOP ( 'NONE', ( #34585, #111945, #32100, #1480 ) ) ;
#12121=ORIENTED_EDGE ( 'NONE', *, *, #6829, .F. ) ;
#12122=DIRECTION ( 'NONE',  ( 0.000000000000000000, 0.000000000000000000, -1.000000000000000000 ) ) ;
#12123=DIRECTION ( 'NONE',  ( -0.000000000000000000, 1.000000000000000000, -0.000000000000000000 ) ) ;
#12124=CARTESIAN_POINT ( 'NONE',  ( 0.3999999999999568345, 2.500000000000000000, -3.637306695894650055 ) ) ;
#12125=CARTESIAN_POINT ( 'NONE',  ( 0.1999999999999567124, 12.50000000000000000, -4.048810130592463530 ) ) ;
#12126=DIRECTION ( 'NONE',  ( 0.000000000000000000, -0.000000000000000000, 1.000000000000000000 ) ) ;
#12127=EDGE_LOOP ( 'NONE', ( #5410, #40025 ) ) ;
#12128=DIRECTION ( 'NONE',  ( 0.000000000000000000, -0.9999939076577903929, 0.003490651415223739937 ) ) ;
#12129=CONICAL_SURFACE ( 'NONE', #78969, 0.09999999999999982514, 0.003490658503988666988 ) ;
#12130=ADVANCED_FACE ( 'NONE', ( #1936 ), #1299, .T. ) ;
#12131=ORIENTED_EDGE ( 'NONE', *, *, #109422, .F. ) ;
#12132=CARTESIAN_POINT ( 'NONE',  ( 17.50000000000000000, 2.499999999999999556, -2.333333333333329485 ) ) ;
#12133=PLANE ( 'NONE',  #106958 ) ;
#12134=DIRECTION ( 'NONE',  ( 0.000000000000000000, 1.000000000000000000, 0.000000000000000000 ) ) ;
#12135=DIRECTION ( 'NONE',  ( 0.000000000000000000, 1.000000000000000000, 0.000000000000000000 ) ) ;
#12136=EDGE_CURVE ( 'NONE', #71261, #30351, #25951, .T. ) ;
#12137=CARTESIAN_POINT ( 'NONE',  ( 8.099999999999923261, 2.500000000000000000, -4.676537180435978769 ) ) ;
#12138=ADVANCED_FACE ( 'NONE', ( #83737 ), #9224, .T. ) ;
#12139=ORIENTED_EDGE ( 'NONE', *, *, #98916, .T. ) ;
#12140=CARTESIAN_POINT ( 'NONE',  ( -3.550000000000027356, 2.500000000000000000, 1.818653347947321475 ) ) ;
#12141=EDGE_CURVE ( 'NONE', #4440, #55939, #53140, .T. ) ;
#12142=LINE ( 'NONE', #72386, #21503 ) ;
#12143=ORIENTED_EDGE ( 'NONE', *, *, #101548, .T. ) ;
#12144=EDGE_CURVE ( 'NONE', #103611, #63897, #41250, .T. ) ;
#12145=ORIENTED_EDGE ( 'NONE', *, *, #67235, .F. ) ;
#12146=VERTEX_POINT ( 'NONE', #71991 ) ;
#12147=DIRECTION ( 'NONE',  ( -4.274815082592931898E-19, -0.9999939076577903929, -0.003490651415223739937 ) ) ;
#12148=FACE_OUTER_BOUND ( 'NONE', #27107, .T. ) ;
#12149=ADVANCED_FACE ( 'NONE', ( #81161 ), #92250, .T. ) ;
#12152=DIRECTION ( 'NONE',  ( 0.000000000000000000, -0.9999939076577903929, 0.003490651415223739937 ) ) ;
#12153=CIRCLE ( 'NONE', #47680, 0.1000000000000002554 ) ;
#12154=FACE_OUTER_BOUND ( 'NONE', #116426, .T. ) ;
#12155=VECTOR ( 'NONE', #36842, 1000.000000000000000 ) ;
#12156=DIRECTION ( 'NONE',  ( -0.000000000000000000, -1.000000000000000000, -0.000000000000000000 ) ) ;
#12157=DIRECTION ( 'NONE',  ( 0.000000000000000000, -0.9999939076577903929, 0.003490651415223739937 ) ) ;
#12158=CARTESIAN_POINT ( 'NONE',  ( 12.04999999999990834, 2.500000000000000000, -2.065063509461102065 ) ) ;
#12159=EDGE_LOOP ( 'NONE', ( #32953, #61186, #119767, #84581 ) ) ;
#12160=DIRECTION ( 'NONE',  ( -0.000000000000000000, -1.000000000000000000, -0.000000000000000000 ) ) ;
#12161=DIRECTION ( 'NONE',  ( 0.000000000000000000, 1.000000000000000000, 0.000000000000000000 ) ) ;
#12162=FACE_OUTER_BOUND ( 'NONE', #58442, .T. ) ;
#12163=DIRECTION ( 'NONE',  ( 0.000000000000000000, -0.000000000000000000, 1.000000000000000000 ) ) ;
#12164=EDGE_LOOP ( 'NONE', ( #58186, #120938, #47158, #39150 ) ) ;
#12165=DIRECTION ( 'NONE',  ( 0.000000000000000000, 0.000000000000000000, -1.000000000000000000 ) ) ;
#12166=AXIS2_PLACEMENT_3D ( 'NONE', #126458, #8580, #101346 ) ;
#12167=VECTOR ( 'NONE', #64195, 1000.000000000000000 ) ;
#12168=DIRECTION ( 'NONE',  ( 0.000000000000000000, 0.000000000000000000, 1.000000000000000000 ) ) ;
#12169=FACE_OUTER_BOUND ( 'NONE', #98085, .T. ) ;
#12170=EDGE_LOOP ( 'NONE', ( #45047, #81907 ) ) ;
#12171=ORIENTED_EDGE ( 'NONE', *, *, #72429, .F. ) ;
#12172=LINE ( 'NONE', #49557, #107407 ) ;
#12173=VERTEX_POINT ( 'NONE', #62176 ) ;
#12174=ORIENTED_EDGE ( 'NONE', *, *, #7889, .T. ) ;
#12175=CARTESIAN_POINT ( 'NONE',  ( -1.850000000000033396, 12.50000000000000000, -2.511473670974877948 ) ) ;
#12176=EDGE_CURVE ( 'NONE', #22314, #47889, #115827, .T. ) ;
#12177=CIRCLE ( 'NONE', #112558, 0.06509327318403745899 ) ;
#12178=ADVANCED_FACE ( 'NONE', ( #22256 ), #109579, .T. ) ;
#12179=CARTESIAN_POINT ( 'NONE',  ( 8.949999999999915801, 2.500000000000000000, -1.918653347947326004 ) ) ;
#12180=DIRECTION ( 'NONE',  ( 0.000000000000000000, 0.000000000000000000, -1.000000000000000000 ) ) ;
#12181=ADVANCED_FACE ( 'NONE', ( #122380 ), #42698, .T. ) ;
#12182=CARTESIAN_POINT ( 'NONE',  ( 10.64999999999990976, 12.50000000000000000, -6.148780366869526226 ) ) ;
#12183=EDGE_LOOP ( 'NONE', ( #19317, #78519, #128891, #67258 ) ) ;
#12184=VECTOR ( 'NONE', #86386, 1000.000000000000000 ) ;
#12185=VECTOR ( 'NONE', #57894, 1000.000000000000000 ) ;
#12186=AXIS2_PLACEMENT_3D ( 'NONE', #25453, #45773, #95503 ) ;
#12187=AXIS2_PLACEMENT_3D ( 'NONE', #117073, #126275, #75872 ) ;
#12188=PLANE ( 'NONE',  #37807 ) ;
#12189=VERTEX_POINT ( 'NONE', #3876 ) ;
#12191=CARTESIAN_POINT ( 'NONE',  ( 17.28959186693766981, 1.567451025700696610, 5.035561754028593739 ) ) ;
#12192=EDGE_CURVE ( 'NONE', #129191, #46687, #122102, .T. ) ;
#12193=CARTESIAN_POINT ( 'NONE',  ( -10.45000000000000462, 2.500000000000000000, -2.265063509461097802 ) ) ;
#12194=CIRCLE ( 'NONE', #56115, 0.06509327318403745899 ) ;
#12195=EDGE_CURVE ( 'NONE', #101934, #106042, #2968, .T. ) ;
#12196=ORIENTED_EDGE ( 'NONE', *, *, #3778, .F. ) ;
#12197=AXIS2_PLACEMENT_3D ( 'NONE', #110657, #70739, #81833 ) ;
#12198=ADVANCED_FACE ( 'NONE', ( #98611 ), #39744, .T. ) ;
#12199=AXIS2_PLACEMENT_3D ( 'NONE', #125676, #41138, #72523 ) ;
#12200=EDGE_CURVE ( 'NONE', #87361, #3965, #49550, .T. ) ;
#12201=ORIENTED_EDGE ( 'NONE', *, *, #102493, .T. ) ;
#12202=ORIENTED_EDGE ( 'NONE', *, *, #9839, .T. ) ;
#12205=CARTESIAN_POINT ( 'NONE',  ( 9.399999999999915090, 12.50000000000000000, 4.741630453620009789 ) ) ;
#12206=CARTESIAN_POINT ( 'NONE',  ( 8.349999999999923261, 2.500000000000000000, -5.702370205355749455 ) ) ;
#12207=FACE_BOUND ( 'NONE', #48689, .T. ) ;
#12208=VERTEX_POINT ( 'NONE', #79017 ) ;
#12209=LINE ( 'NONE', #53918, #41183 ) ;
#12211=EDGE_CURVE ( 'NONE', #115574, #98477, #119550, .T. ) ;
#12212=CIRCLE ( 'NONE', #3814, 0.1000000000000000472 ) ;
#12213=CARTESIAN_POINT ( 'NONE',  ( -6.249999999999981348, 2.500000000000000000, 6.595190528383296780 ) ) ;
#12214=DIRECTION ( 'NONE',  ( 0.000000000000000000, 0.000000000000000000, -1.000000000000000000 ) ) ;
#12215=AXIS2_PLACEMENT_3D ( 'NONE', #31491, #51144, #111307 ) ;
#12217=DIRECTION ( 'NONE',  ( 0.000000000000000000, 0.000000000000000000, 1.000000000000000000 ) ) ;
#12218=PLANE ( 'NONE',  #34542 ) ;
#12219=AXIS2_PLACEMENT_3D ( 'NONE', #94202, #104028, #43838 ) ;
#12220=CARTESIAN_POINT ( 'NONE',  ( 7.699999999999922018, 2.500000000000000000, 0.4464101615137735513 ) ) ;
#12221=VERTEX_POINT ( 'NONE', #80294 ) ;
#12222=ORIENTED_EDGE ( 'NONE', *, *, #83713, .F. ) ;
#12223=ORIENTED_EDGE ( 'NONE', *, *, #65859, .F. ) ;
#12225=EDGE_LOOP ( 'NONE', ( #96686, #57614, #127402, #42411 ) ) ;
#12226=ORIENTED_EDGE ( 'NONE', *, *, #22663, .F. ) ;
#12227=AXIS2_PLACEMENT_3D ( 'NONE', #67525, #106815, #66895 ) ;
#12228=DIRECTION ( 'NONE',  ( -0.000000000000000000, 1.000000000000000000, -0.000000000000000000 ) ) ;
#12229=DIRECTION ( 'NONE',  ( 0.000000000000000000, -0.000000000000000000, 1.000000000000000000 ) ) ;
#12230=ORIENTED_EDGE ( 'NONE', *, *, #40144, .F. ) ;
#12231=FACE_BOUND ( 'NONE', #78305, .T. ) ;
#12232=CARTESIAN_POINT ( 'NONE',  ( 10.19999999999991225, 2.500000000000000000, -4.676537180435978769 ) ) ;
#12233=AXIS2_PLACEMENT_3D ( 'NONE', #118406, #98118, #119061 ) ;
#12234=VERTEX_POINT ( 'NONE', #58713 ) ;
#12235=DIRECTION ( 'NONE',  ( 0.000000000000000000, 0.000000000000000000, -1.000000000000000000 ) ) ;
#12236=DIRECTION ( 'NONE',  ( 0.000000000000000000, -0.9999939076577903929, 0.003490651415223739937 ) ) ;
#12237=DIRECTION ( 'NONE',  ( 0.000000000000000000, -0.000000000000000000, 1.000000000000000000 ) ) ;
#12238=ORIENTED_EDGE ( 'NONE', *, *, #25147, .T. ) ;
#12239=AXIS2_PLACEMENT_3D ( 'NONE', #60614, #70415, #61245 ) ;
#12240=LINE ( 'NONE', #101285, #95267 ) ;
#12241=AXIS2_PLACEMENT_3D ( 'NONE', #32190, #59718, #72738 ) ;
#12242=ORIENTED_EDGE ( 'NONE', *, *, #40430, .T. ) ;
#12243=EDGE_CURVE ( 'NONE', #118050, #102673, #29265, .T. ) ;
#12244=EDGE_LOOP ( 'NONE', ( #43384, #45348, #55426, #88169 ) ) ;
#12245=VERTEX_POINT ( 'NONE', #57430 ) ;
#12246=DIRECTION ( 'NONE',  ( 0.000000000000000000, 0.000000000000000000, 1.000000000000000000 ) ) ;
#12247=CARTESIAN_POINT ( 'NONE',  ( -11.24999999999996447, 2.500000000000000000, -6.495190528383298911 ) ) ;
#12248=VECTOR ( 'NONE', #70221, 1000.000000000000000 ) ;
#12249=EDGE_LOOP ( 'NONE', ( #5801, #6411, #118499, #111658 ) ) ;
#12250=CARTESIAN_POINT ( 'NONE',  ( -5.650000000000023448, 2.500000000000000000, -1.718653347947326049 ) ) ;
#12251=DIRECTION ( 'NONE',  ( -0.000000000000000000, 1.000000000000000000, -0.000000000000000000 ) ) ;
#12252=CARTESIAN_POINT ( 'NONE',  ( 12.49999999999990408, 2.500000000000000000, 5.022947341949748790 ) ) ;
#12253=CARTESIAN_POINT ( 'NONE',  ( -12.49999999999995737, 2.500000000000000000, 4.330127018922196314 ) ) ;
#12254=AXIS2_PLACEMENT_3D ( 'NONE', #103495, #34770, #64842 ) ;
#12256=ORIENTED_EDGE ( 'NONE', *, *, #6353, .F. ) ;
#12257=AXIS2_PLACEMENT_3D ( 'NONE', #3707, #85497, #72464 ) ;
#12258=EDGE_CURVE ( 'NONE', #109879, #32296, #38447, .T. ) ;
#12259=LINE ( 'NONE', #92110, #62114 ) ;
#12260=ORIENTED_EDGE ( 'NONE', *, *, #91246, .F. ) ;
#12261=CARTESIAN_POINT ( 'NONE',  ( 1.649999999999949729, 2.500000000000000000, 7.188010851410848723 ) ) ;
#12262=AXIS2_PLACEMENT_3D ( 'NONE', #88156, #38460, #57443 ) ;
#12263=VERTEX_POINT ( 'NONE', #70464 ) ;
#12264=CARTESIAN_POINT ( 'NONE',  ( -11.24999999999999822, 2.500000000000000000, 1.572243186433545548 ) ) ;
#12265=ORIENTED_EDGE ( 'NONE', *, *, #39128, .T. ) ;
#12266=DIRECTION ( 'NONE',  ( -0.000000000000000000, -1.000000000000000000, -0.000000000000000000 ) ) ;
#12267=CARTESIAN_POINT ( 'NONE',  ( -2.100000000000034284, 2.500000000000000000, -4.330127018922201643 ) ) ;
#12268=DIRECTION ( 'NONE',  ( -0.000000000000000000, -1.000000000000000000, -0.000000000000000000 ) ) ;
#12269=DIRECTION ( 'NONE',  ( 0.000000000000000000, 0.000000000000000000, 1.000000000000000000 ) ) ;
#12270=CARTESIAN_POINT ( 'NONE',  ( -6.900000000000019007, 12.50000000000000000, 0.2813168883297361700 ) ) ;
#12271=ORIENTED_EDGE ( 'NONE', *, *, #85320, .F. ) ;
#12272=ORIENTED_EDGE ( 'NONE', *, *, #82485, .T. ) ;
#12274=CARTESIAN_POINT ( 'NONE',  ( 3.149999999999946176, 12.50000000000000000, -2.511473670974877948 ) ) ;
#12275=CARTESIAN_POINT ( 'NONE',  ( 8.949999999999917577, 2.500000000000000000, -2.511473670974877948 ) ) ;
#12276=CONICAL_SURFACE ( 'NONE', #60438, 0.1000000000000000472, 0.003490658503988666988 ) ;
#12277=ORIENTED_EDGE ( 'NONE', *, *, #11583, .T. ) ;
#12278=EDGE_LOOP ( 'NONE', ( #77660, #94393 ) ) ;
#12279=ORIENTED_EDGE ( 'NONE', *, *, #97135, .F. ) ;
#12280=CARTESIAN_POINT ( 'NONE',  ( -10.00000000000000533, 12.50000000000000000, 5.022947341949748790 ) ) ;
#12281=ORIENTED_EDGE ( 'NONE', *, *, #101009, .T. ) ;
#12282=DIRECTION ( 'NONE',  ( 0.000000000000000000, 0.000000000000000000, -1.000000000000000000 ) ) ;
#12283=CARTESIAN_POINT ( 'NONE',  ( 2.699999999999944666, 12.50000000000000000, 4.741630453620009789 ) ) ;
#12284=CIRCLE ( 'NONE', #66655, 0.06509327318403745899 ) ;
#12285=EDGE_CURVE ( 'NONE', #331, #91012, #56756, .T. ) ;
#12286=AXIS2_PLACEMENT_3D ( 'NONE', #101025, #40183, #49373 ) ;
#12287=CARTESIAN_POINT ( 'NONE',  ( -5.850000000000022737, 12.50000000000000000, -2.165063509461101710 ) ) ;
#12288=ORIENTED_EDGE ( 'NONE', *, *, #6779, .T. ) ;
#12289=DIRECTION ( 'NONE',  ( 0.000000000000000000, 1.000000000000000000, 0.000000000000000000 ) ) ;
#12290=VECTOR ( 'NONE', #26626, 1000.000000000000000 ) ;
#12291=DIRECTION ( 'NONE',  ( -0.000000000000000000, 1.000000000000000000, -0.000000000000000000 ) ) ;
#12292=DIRECTION ( 'NONE',  ( -0.000000000000000000, 1.000000000000000000, -0.000000000000000000 ) ) ;
#12293=CARTESIAN_POINT ( 'NONE',  ( 14.14999999999989733, 12.50000000000000000, 2.857883832488649301 ) ) ;
#12294=DIRECTION ( 'NONE',  ( 0.000000000000000000, 0.000000000000000000, 1.000000000000000000 ) ) ;
#12295=EDGE_CURVE ( 'NONE', #48486, #20699, #59385, .T. ) ;
#12296=CONICAL_SURFACE ( 'NONE', #100144, 0.09999999999999982514, 0.003490658503988666988 ) ;
#12297=ORIENTED_EDGE ( 'NONE', *, *, #4938, .F. ) ;
#12298=AXIS2_PLACEMENT_3D ( 'NONE', #30032, #22152, #62069 ) ;
#12299=DIRECTION ( 'NONE',  ( 0.000000000000000000, -0.9999939076577903929, 0.003490651415223739937 ) ) ;
#12300=CARTESIAN_POINT ( 'NONE',  ( 43.06166283080823831, -3.066941195843063017, 4.904920240851240010 ) ) ;
#12301=EDGE_CURVE ( 'NONE', #59954, #59797, #109753, .T. ) ;
#12302=EDGE_LOOP ( 'NONE', ( #51723, #15027 ) ) ;
#12303=EDGE_CURVE ( 'NONE', #43630, #54835, #14891, .T. ) ;
#12304=ORIENTED_EDGE ( 'NONE', *, *, #54398, .T. ) ;
#12305=EDGE_CURVE ( 'NONE', #35208, #50586, #50515, .T. ) ;
#12307=CARTESIAN_POINT ( 'NONE',  ( -12.04999999999999716, 2.500000000000000000, -6.495190528383298911 ) ) ;
#12308=EDGE_CURVE ( 'NONE', #127093, #86483, #94330, .T. ) ;
#12309=ADVANCED_FACE ( 'NONE', ( #99290 ), #9609, .T. ) ;
#12310=CARTESIAN_POINT ( 'NONE',  ( -5.850000000000021849, 12.50000000000000000, -5.802370205355749988 ) ) ;
#12311=CIRCLE ( 'NONE', #56217, 0.09999999999999982514 ) ;
#12312=DIRECTION ( 'NONE',  ( 0.000000000000000000, 1.000000000000000000, 0.000000000000000000 ) ) ;
#12313=CARTESIAN_POINT ( 'NONE',  ( -12.09999999999999609, 2.500000000000000000, 0.6928203230275535862 ) ) ;
#12314=CONICAL_SURFACE ( 'NONE', #68749, 0.1000000000000002554, 0.003490658503988666988 ) ;
#12315=CARTESIAN_POINT ( 'NONE',  ( -3.150000000000029221, 2.500000000000000000, -1.918653347947326004 ) ) ;
#12316=DIRECTION ( 'NONE',  ( 0.000000000000000000, 0.000000000000000000, 1.000000000000000000 ) ) ;
#12317=CARTESIAN_POINT ( 'NONE',  ( -12.94999999999999218, 2.500000000000000000, 2.065063509461101621 ) ) ;
#12318=ADVANCED_FACE ( 'NONE', ( #89460 ), #42127, .T. ) ;
#12319=CARTESIAN_POINT ( 'NONE',  ( 2.499999999999948930, 12.50000000000000000, -0.6928203230275541413 ) ) ;
#12320=EDGE_CURVE ( 'NONE', #45894, #11512, #10788, .T. ) ;
#12321=AXIS2_PLACEMENT_3D ( 'NONE', #24511, #125290, #95825 ) ;
#12322=ORIENTED_EDGE ( 'NONE', *, *, #64793, .F. ) ;
#12323=EDGE_CURVE ( 'NONE', #124247, #101388, #118268, .T. ) ;
#12324=ORIENTED_EDGE ( 'NONE', *, *, #43148, .T. ) ;
#12325=ORIENTED_EDGE ( 'NONE', *, *, #66981, .F. ) ;
#12326=AXIS2_PLACEMENT_3D ( 'NONE', #102171, #70772, #91057 ) ;
#12327=VERTEX_POINT ( 'NONE', #48245 ) ;
#12328=CARTESIAN_POINT ( 'NONE',  ( 15.79999999999989058, 2.500000000000000000, 0.09999999999999761857 ) ) ;
#12330=ORIENTED_EDGE ( 'NONE', *, *, #100279, .F. ) ;
#12331=CARTESIAN_POINT ( 'NONE',  ( -1.250000000000037526, 2.500000000000000000, -1.572243186433550211 ) ) ;
#12332=CIRCLE ( 'NONE', #39565, 0.06509327318403745899 ) ;
#12333=DIRECTION ( 'NONE',  ( 0.000000000000000000, 1.000000000000000000, 0.000000000000000000 ) ) ;
#12334=LINE ( 'NONE', #96678, #7823 ) ;
#12335=EDGE_LOOP ( 'NONE', ( #125447, #104878, #93490, #60054 ) ) ;
#12336=CARTESIAN_POINT ( 'NONE',  ( -12.29999999999999716, 2.500000000000000000, -3.883716857408423984 ) ) ;
#12337=CIRCLE ( 'NONE', #54113, 0.1000000000000000472 ) ;
#12338=FACE_OUTER_BOUND ( 'NONE', #44546, .T. ) ;
#12339=EDGE_LOOP ( 'NONE', ( #126212, #81232, #101910, #13754 ) ) ;
#12340=VECTOR ( 'NONE', #90264, 1000.000000000000000 ) ;
#12341=VERTEX_POINT ( 'NONE', #68523 ) ;
#12342=EDGE_LOOP ( 'NONE', ( #30328, #114813 ) ) ;
#12343=ORIENTED_EDGE ( 'NONE', *, *, #94660, .T. ) ;
#12344=CARTESIAN_POINT ( 'NONE',  ( -10.85000000000000142, 2.500000000000000000, 6.495190528383297135 ) ) ;
#12345=VECTOR ( 'NONE', #12740, 1000.000000000000000 ) ;
#12346=CARTESIAN_POINT ( 'NONE',  ( 1.699999999999951994, 2.500000000000000000, 0.09999999999999772959 ) ) ;
#12347=DIRECTION ( 'NONE',  ( 0.000000000000000000, 1.000000000000000000, 0.000000000000000000 ) ) ;
#12348=EDGE_CURVE ( 'NONE', #65138, #74205, #17029, .T. ) ;
#12349=CARTESIAN_POINT ( 'NONE',  ( 2.949999999999946887, 12.50000000000000000, -6.430097255199264339 ) ) ;
#12351=EDGE_CURVE ( 'NONE', #2207, #65686, #125717, .T. ) ;
#12352=AXIS2_PLACEMENT_3D ( 'NONE', #16853, #98657, #85627 ) ;
#12353=PLANE ( 'NONE',  #85731 ) ;
#12354=ORIENTED_EDGE ( 'NONE', *, *, #66517, .F. ) ;
#12355=CARTESIAN_POINT ( 'NONE',  ( -2.050000000000033129, 2.500000000000000000, 6.595190528383296780 ) ) ;
#12356=CARTESIAN_POINT ( 'NONE',  ( -2.700000000000030376, 2.500000000000000000, 3.883716857408421319 ) ) ;
#12357=CIRCLE ( 'NONE', #118971, 0.1000000000000002554 ) ;
#12358=CARTESIAN_POINT ( 'NONE',  ( -11.25000000000000000, 12.50000000000000000, -7.188010851410850499 ) ) ;
#12359=DIRECTION ( 'NONE',  ( 0.000000000000000000, 0.000000000000000000, 1.000000000000000000 ) ) ;
#12360=EDGE_CURVE ( 'NONE', #48711, #46223, #121518, .T. ) ;
#12361=ADVANCED_FACE ( 'NONE', ( #12169 ), #102744, .T. ) ;
#12362=EDGE_LOOP ( 'NONE', ( #77210, #25191 ) ) ;
#12363=CIRCLE ( 'NONE', #4041, 0.1000000000000002554 ) ;
#12364=AXIS2_PLACEMENT_3D ( 'NONE', #34439, #93987, #64514 ) ;
#12365=EDGE_CURVE ( 'NONE', #102047, #128215, #51481, .T. ) ;
#12366=VERTEX_POINT ( 'NONE', #52749 ) ;
#12367=ORIENTED_EDGE ( 'NONE', *, *, #82068, .F. ) ;
#12368=DIRECTION ( 'NONE',  ( -0.000000000000000000, 1.000000000000000000, -0.000000000000000000 ) ) ;
#12369=DIRECTION ( 'NONE',  ( 0.000000000000000000, 1.000000000000000000, 0.000000000000000000 ) ) ;
#12370=CARTESIAN_POINT ( 'NONE',  ( -6.650000000000014566, 12.50000000000000000, 2.165063509461097713 ) ) ;
#12371=FACE_BOUND ( 'NONE', #59041, .T. ) ;
#12372=DIRECTION ( 'NONE',  ( 0.000000000000000000, 1.000000000000000000, 0.000000000000000000 ) ) ;
#12373=DIRECTION ( 'NONE',  ( 0.000000000000000000, 0.000000000000000000, 1.000000000000000000 ) ) ;
#12374=ADVANCED_FACE ( 'NONE', ( #110383 ), #109000, .T. ) ;
#12375=PLANE ( 'NONE',  #33220 ) ;
#12376=VECTOR ( 'NONE', #56518, 1000.000000000000000 ) ;
#12377=DIRECTION ( 'NONE',  ( 0.000000000000000000, 1.000000000000000000, 0.000000000000000000 ) ) ;
#12378=DIRECTION ( 'NONE',  ( -0.000000000000000000, -1.000000000000000000, -0.000000000000000000 ) ) ;
#12379=DIRECTION ( 'NONE',  ( -4.274815082592931898E-19, -0.9999939076577903929, -0.003490651415223739937 ) ) ;
#12380=VERTEX_POINT ( 'NONE', #42300 ) ;
#12381=CARTESIAN_POINT ( 'NONE',  ( -2.950000000000029932, 2.500000000000000000, 2.165063509461097713 ) ) ;
#12382=CIRCLE ( 'NONE', #100220, 0.06509327318403745899 ) ;
#12383=AXIS2_PLACEMENT_3D ( 'NONE', #42448, #41812, #1852 ) ;
#12384=CARTESIAN_POINT ( 'NONE',  ( 6.449999999999930012, 12.50000000000000000, 6.841600689897072485 ) ) ;
#12385=ORIENTED_EDGE ( 'NONE', *, *, #65125, .T. ) ;
#12386=EDGE_LOOP ( 'NONE', ( #49177, #87405, #77813, #75221 ) ) ;
#12387=DIRECTION ( 'NONE',  ( -0.000000000000000000, 1.000000000000000000, -0.000000000000000000 ) ) ;
#12388=CARTESIAN_POINT ( 'NONE',  ( 2.099999999999950351, 2.500000000000000000, -4.230127018922201998 ) ) ;
#12389=EDGE_CURVE ( 'NONE', #112381, #43111, #69293, .T. ) ;
#12390=FACE_BOUND ( 'NONE', #87461, .T. ) ;
#12391=DIRECTION ( 'NONE',  ( 0.000000000000000000, 0.000000000000000000, 1.000000000000000000 ) ) ;
#12392=AXIS2_PLACEMENT_3D ( 'NONE', #21853, #33599, #4109 ) ;
#12393=AXIS2_PLACEMENT_3D ( 'NONE', #12436, #91013, #51105 ) ;
#12394=ORIENTED_EDGE ( 'NONE', *, *, #51603, .T. ) ;
#12395=FACE_OUTER_BOUND ( 'NONE', #39766, .T. ) ;
#12397=ORIENTED_EDGE ( 'NONE', *, *, #6340, .F. ) ;
#12398=DIRECTION ( 'NONE',  ( 0.000000000000000000, 0.000000000000000000, 1.000000000000000000 ) ) ;
#12399=CARTESIAN_POINT ( 'NONE',  ( -4.200000000000025935, 2.500000000000000000, 4.330127018922196314 ) ) ;
#12400=AXIS2_PLACEMENT_3D ( 'NONE', #42806, #13943, #93811 ) ;
#12401=CIRCLE ( 'NONE', #68846, 0.09999999999999982514 ) ;
#12402=ADVANCED_FACE ( 'NONE', ( #120853 ), #81819, .T. ) ;
#12403=VERTEX_POINT ( 'NONE', #80939 ) ;
#12404=DIRECTION ( 'NONE',  ( 0.000000000000000000, 1.000000000000000000, 0.000000000000000000 ) ) ;
#12405=CARTESIAN_POINT ( 'NONE',  ( -1.050000000000037348, 2.500000000000000000, -6.841600689897078702 ) ) ;
#12408=DIRECTION ( 'NONE',  ( 0.000000000000000000, 0.000000000000000000, -1.000000000000000000 ) ) ;
#12409=CARTESIAN_POINT ( 'NONE',  ( -3.550000000000027800, 12.50000000000000000, 6.148780366869520009 ) ) ;
#12410=VECTOR ( 'NONE', #8939, 1000.000000000000000 ) ;
#12411=ORIENTED_EDGE ( 'NONE', *, *, #62462, .F. ) ;
#12412=ORIENTED_EDGE ( 'NONE', *, *, #53378, .T. ) ;
#12413=EDGE_CURVE ( 'NONE', #126865, #76363, #6571, .T. ) ;
#12414=DIRECTION ( 'NONE',  ( -0.000000000000000000, 1.000000000000000000, -0.000000000000000000 ) ) ;
#12415=VERTEX_POINT ( 'NONE', #121480 ) ;
#12416=DIRECTION ( 'NONE',  ( -4.274815082592931898E-19, -0.9999939076577903929, -0.003490651415223739937 ) ) ;
#12417=DIRECTION ( 'NONE',  ( -0.000000000000000000, -1.000000000000000000, -0.000000000000000000 ) ) ;
#12418=DIRECTION ( 'NONE',  ( 0.000000000000000000, 0.000000000000000000, 1.000000000000000000 ) ) ;
#12419=ORIENTED_EDGE ( 'NONE', *, *, #78521, .F. ) ;
#12420=CARTESIAN_POINT ( 'NONE',  ( 7.499999999999960032, 2.500000000000000000, -2.276824562219559311E-15 ) ) ;
#12421=CARTESIAN_POINT ( 'NONE',  ( -1.250000000000037526, 2.500000000000000000, -5.802370205355749988 ) ) ;
#12422=DIRECTION ( 'NONE',  ( -0.000000000000000000, 1.000000000000000000, -0.000000000000000000 ) ) ;
#12423=CARTESIAN_POINT ( 'NONE',  ( -10.40000000000000213, 2.500000000000000000, 3.637306695894644726 ) ) ;
#12424=CARTESIAN_POINT ( 'NONE',  ( -6.850000000000013856, 12.50000000000000000, 2.511473670974873507 ) ) ;
#12425=AXIS2_PLACEMENT_3D ( 'NONE', #102936, #11977, #2156 ) ;
#12426=DIRECTION ( 'NONE',  ( 0.000000000000000000, 0.000000000000000000, 1.000000000000000000 ) ) ;
#12427=ORIENTED_EDGE ( 'NONE', *, *, #91682, .F. ) ;
#12428=VERTEX_POINT ( 'NONE', #82220 ) ;
#12429=CARTESIAN_POINT ( 'NONE',  ( -9.800000000000004263, 12.50000000000000000, -0.4115034346978157509 ) ) ;
#12430=ORIENTED_EDGE ( 'NONE', *, *, #90568, .F. ) ;
#12432=ORIENTED_EDGE ( 'NONE', *, *, #105907, .F. ) ;
#12433=EDGE_LOOP ( 'NONE', ( #23643, #62641 ) ) ;
#12434=ORIENTED_EDGE ( 'NONE', *, *, #41877, .T. ) ;
#12435=AXIS2_PLACEMENT_3D ( 'NONE', #98396, #86655, #48676 ) ;
#12436=CARTESIAN_POINT ( 'NONE',  ( 13.34999999999990017, 2.500000000000000000, 2.165063509461097713 ) ) ;
#12437=DIRECTION ( 'NONE',  ( 0.000000000000000000, -0.000000000000000000, 1.000000000000000000 ) ) ;
#12438=DIRECTION ( 'NONE',  ( 0.000000000000000000, 0.000000000000000000, -1.000000000000000000 ) ) ;
#12439=ADVANCED_FACE ( 'NONE', ( #32503 ), #35862, .T. ) ;
#12440=AXIS2_PLACEMENT_3D ( 'NONE', #81566, #129411, #22662 ) ;
#12441=CIRCLE ( 'NONE', #83482, 0.1000000000000000472 ) ;
#12442=DIRECTION ( 'NONE',  ( -0.000000000000000000, -1.000000000000000000, -0.000000000000000000 ) ) ;
#12443=CARTESIAN_POINT ( 'NONE',  ( 12.49999999999993960, 12.50000000000000000, -4.330127018922201643 ) ) ;
#12444=DIRECTION ( 'NONE',  ( 0.000000000000000000, -0.000000000000000000, 1.000000000000000000 ) ) ;
#12445=LINE ( 'NONE', #121759, #53903 ) ;
#12446=DIRECTION ( 'NONE',  ( -4.274815082592931898E-19, -0.9999939076577903929, -0.003490651415223739937 ) ) ;
#12447=CIRCLE ( 'NONE', #22935, 0.1000000000000000472 ) ;
#12448=DIRECTION ( 'NONE',  ( 0.000000000000000000, 1.000000000000000000, 0.000000000000000000 ) ) ;
#12449=EDGE_CURVE ( 'NONE', #39786, #49438, #111046, .T. ) ;
#12450=CIRCLE ( 'NONE', #58444, 0.09999999999999982514 ) ;
#12451=AXIS2_PLACEMENT_3D ( 'NONE', #105743, #125381, #45542 ) ;
#12452=ORIENTED_EDGE ( 'NONE', *, *, #87307, .F. ) ;
#12453=CARTESIAN_POINT ( 'NONE',  ( -4.400000000000028777, 2.500000000000000000, -3.983716857408426293 ) ) ;
#12454=EDGE_CURVE ( 'NONE', #114896, #57762, #12844, .T. ) ;
#12455=ORIENTED_EDGE ( 'NONE', *, *, #96496, .T. ) ;
#12456=EDGE_CURVE ( 'NONE', #26773, #40065, #113209, .T. ) ;
#12457=ORIENTED_EDGE ( 'NONE', *, *, #56393, .T. ) ;
#12458=EDGE_CURVE ( 'NONE', #44264, #110118, #53410, .T. ) ;
#12459=DIRECTION ( 'NONE',  ( -0.000000000000000000, -1.000000000000000000, -0.000000000000000000 ) ) ;
#12460=CARTESIAN_POINT ( 'NONE',  ( -7.900000000000011013, 2.500000000000000000, 5.022947341949748790 ) ) ;
#12461=EDGE_CURVE ( 'NONE', #22628, #42741, #1072, .T. ) ;
#12462=DIRECTION ( 'NONE',  ( 0.000000000000000000, 0.000000000000000000, 1.000000000000000000 ) ) ;
#12463=DIRECTION ( 'NONE',  ( 0.000000000000000000, 0.000000000000000000, 1.000000000000000000 ) ) ;
#12464=DIRECTION ( 'NONE',  ( 0.000000000000000000, 1.000000000000000000, 0.000000000000000000 ) ) ;
#12465=CARTESIAN_POINT ( 'NONE',  ( 8.549999999999920774, 12.50000000000000000, -2.511473670974877948 ) ) ;
#12466=EDGE_CURVE ( 'NONE', #78026, #125196, #101217, .T. ) ;
#12467=CARTESIAN_POINT ( 'NONE',  ( -9.150000000000009237, 2.500000000000000000, 2.957883832488649389 ) ) ;
#12468=CIRCLE ( 'NONE', #125347, 0.06509327318403741736 ) ;
#12469=VERTEX_POINT ( 'NONE', #31203 ) ;
#12470=EDGE_CURVE ( 'NONE', #3256, #50948, #71106, .T. ) ;
#12471=EDGE_CURVE ( 'NONE', #2782, #85021, #21360, .T. ) ;
#12472=EDGE_CURVE ( 'NONE', #126669, #92740, #91386, .T. ) ;
#12473=ORIENTED_EDGE ( 'NONE', *, *, #105276, .F. ) ;
#12474=AXIS2_PLACEMENT_3D ( 'NONE', #104283, #42814, #102359 ) ;
#12475=EDGE_CURVE ( 'NONE', #123277, #56997, #33799, .T. ) ;
#12476=VECTOR ( 'NONE', #4405, 1000.000000000000000 ) ;
#12477=VERTEX_POINT ( 'NONE', #125362 ) ;
#12478=EDGE_LOOP ( 'NONE', ( #62090, #19174 ) ) ;
#12479=ORIENTED_EDGE ( 'NONE', *, *, #90400, .T. ) ;
#12480=EDGE_CURVE ( 'NONE', #942, #27571, #106948, .T. ) ;
#12481=CARTESIAN_POINT ( 'NONE',  ( 0.3999999999999568345, 2.500000000000000000, -5.122947341949753763 ) ) ;
#12482=CONICAL_SURFACE ( 'NONE', #85646, 0.1000000000000002554, 0.003490658503988666988 ) ;
#12483=CARTESIAN_POINT ( 'NONE',  ( -2.700000000000030820, 2.500000000000000000, -4.083716857408426826 ) ) ;
#12484=CONICAL_SURFACE ( 'NONE', #102380, 0.09999999999999999167, 0.003490658503988666988 ) ;
#12485=CIRCLE ( 'NONE', #14530, 0.1000000000000002554 ) ;
#12486=DIRECTION ( 'NONE',  ( -4.274815082592931898E-19, -0.9999939076577903929, -0.003490651415223739937 ) ) ;
#12487=LINE ( 'NONE', #21678, #46826 ) ;
#12488=PLANE ( 'NONE',  #15784 ) ;
#12489=VERTEX_POINT ( 'NONE', #73672 ) ;
#12490=DIRECTION ( 'NONE',  ( 0.000000000000000000, 0.000000000000000000, -1.000000000000000000 ) ) ;
#12491=DIRECTION ( 'NONE',  ( 0.000000000000000000, 0.000000000000000000, 1.000000000000000000 ) ) ;
#12492=DIRECTION ( 'NONE',  ( -4.274815082592931898E-19, -0.9999939076577903929, -0.003490651415223739937 ) ) ;
#12493=CARTESIAN_POINT ( 'NONE',  ( 3.549999999999941203, 2.500000000000000000, 6.148780366869520897 ) ) ;
#12494=AXIS2_PLACEMENT_3D ( 'NONE', #78742, #36228, #118633 ) ;
#12496=AXIS2_PLACEMENT_3D ( 'NONE', #126494, #67541, #16511 ) ;
#12497=ORIENTED_EDGE ( 'NONE', *, *, #42204, .F. ) ;
#12498=VERTEX_POINT ( 'NONE', #56601 ) ;
#12499=ORIENTED_EDGE ( 'NONE', *, *, #104214, .T. ) ;
#12500=CARTESIAN_POINT ( 'NONE',  ( 7.899999999999924860, 2.500000000000000000, 5.122947341949749323 ) ) ;
#12501=ORIENTED_EDGE ( 'NONE', *, *, #89431, .F. ) ;
#12502=DIRECTION ( 'NONE',  ( 0.000000000000000000, 0.000000000000000000, -1.000000000000000000 ) ) ;
#12504=CONICAL_SURFACE ( 'NONE', #71015, 0.1000000000000002554, 0.003490658503988666988 ) ;
#12505=ORIENTED_EDGE ( 'NONE', *, *, #46421, .T. ) ;
#12506=CARTESIAN_POINT ( 'NONE',  ( 7.099999999999925926, 12.50000000000000000, 0.6928203230275494784 ) ) ;
#12507=CARTESIAN_POINT ( 'NONE',  ( -3.750000000000029310, 2.500000000000000000, -7.088010851410853519 ) ) ;
#12508=DIRECTION ( 'NONE',  ( 0.000000000000000000, 1.000000000000000000, 0.000000000000000000 ) ) ;
#12509=DIRECTION ( 'NONE',  ( 0.000000000000000000, 0.000000000000000000, 1.000000000000000000 ) ) ;
#12510=ADVANCED_FACE ( 'NONE', ( #14734 ), #117396, .T. ) ;
#12511=DIRECTION ( 'NONE',  ( 0.000000000000000000, -0.9999939076577903929, 0.003490651415223739937 ) ) ;
#12512=EDGE_CURVE ( 'NONE', #18199, #114810, #74331, .T. ) ;
#12513=VERTEX_POINT ( 'NONE', #116174 ) ;
#12514=ORIENTED_EDGE ( 'NONE', *, *, #66318, .T. ) ;
#12516=CARTESIAN_POINT ( 'NONE',  ( -9.400000000000007461, 2.500000000000000000, -0.3464101615137783474 ) ) ;
#12517=CARTESIAN_POINT ( 'NONE',  ( 9.199999999999915801, 2.500000000000000000, -4.430127018922202176 ) ) ;
#12518=ADVANCED_FACE ( 'NONE', ( #25212 ), #105729, .T. ) ;
#12519=CARTESIAN_POINT ( 'NONE',  ( 8.749999999999920064, 2.500000000000000000, -2.957883832488653830 ) ) ;
#12520=VERTEX_POINT ( 'NONE', #35701 ) ;
#12522=ORIENTED_EDGE ( 'NONE', *, *, #1805, .T. ) ;
#12523=CARTESIAN_POINT ( 'NONE',  ( -7.900000000000014566, 2.500000000000000000, -3.537306695894649966 ) ) ;
#12524=CIRCLE ( 'NONE', #27197, 0.1000000000000002554 ) ;
#12525=CARTESIAN_POINT ( 'NONE',  ( -4.150000000000024336, 12.50000000000000000, 1.472243186433545459 ) ) ;
#12526=CARTESIAN_POINT ( 'NONE',  ( 8.949999999999915801, 12.50000000000000000, 6.841600689897072485 ) ) ;
#12527=CARTESIAN_POINT ( 'NONE',  ( 0.4499999999999569344, 12.50000000000000000, 2.165063509461097713 ) ) ;
#12528=ORIENTED_EDGE ( 'NONE', *, *, #71468, .T. ) ;
#12529=DIRECTION ( 'NONE',  ( 0.000000000000000000, 0.000000000000000000, 1.000000000000000000 ) ) ;
#12530=AXIS2_PLACEMENT_3D ( 'NONE', #26517, #66429, #18623 ) ;
#12531=VECTOR ( 'NONE', #83558, 1000.000000000000000 ) ;
#12532=DIRECTION ( 'NONE',  ( 0.000000000000000000, 0.000000000000000000, 1.000000000000000000 ) ) ;
#12533=ORIENTED_EDGE ( 'NONE', *, *, #60509, .F. ) ;
#12534=LINE ( 'NONE', #80655, #117965 ) ;
#12535=ORIENTED_EDGE ( 'NONE', *, *, #103438, .T. ) ;
#12536=CARTESIAN_POINT ( 'NONE',  ( 4.999999999999935163, 12.50000000000000000, 0.7579135962115869374 ) ) ;
#12537=CIRCLE ( 'NONE', #10483, 0.1000000000000002554 ) ;
#12538=ORIENTED_EDGE ( 'NONE', *, *, #29185, .T. ) ;
#12539=CARTESIAN_POINT ( 'NONE',  ( 8.749999999999921840, 2.500000000000000000, -5.902370205355750521 ) ) ;
#12540=DIRECTION ( 'NONE',  ( 0.000000000000000000, 0.000000000000000000, 1.000000000000000000 ) ) ;
#12541=ORIENTED_EDGE ( 'NONE', *, *, #11567, .T. ) ;
#12542=VERTEX_POINT ( 'NONE', #34427 ) ;
#12543=DIRECTION ( 'NONE',  ( 0.000000000000000000, 0.000000000000000000, -1.000000000000000000 ) ) ;
#12544=LINE ( 'NONE', #121864, #24709 ) ;
#12545=CARTESIAN_POINT ( 'NONE',  ( -4.600000000000024514, 2.500000000000000000, 3.637306695894644726 ) ) ;
#12546=EDGE_CURVE ( 'NONE', #4198, #41152, #125993, .T. ) ;
#12548=LINE ( 'NONE', #70839, #95480 ) ;
#12549=DIRECTION ( 'NONE',  ( -4.274815082592931898E-19, -0.9999939076577903929, -0.003490651415223739937 ) ) ;
#12550=DIRECTION ( 'NONE',  ( -4.274815082592931898E-19, -0.9999939076577903929, -0.003490651415223739937 ) ) ;
#12551=CARTESIAN_POINT ( 'NONE',  ( 2.099999999999947686, 12.50000000000000000, 5.088040615133786027 ) ) ;
#12552=FACE_OUTER_BOUND ( 'NONE', #22893, .T. ) ;
#12553=AXIS2_PLACEMENT_3D ( 'NONE', #9377, #36910, #17893 ) ;
#12554=ORIENTED_EDGE ( 'NONE', *, *, #79038, .F. ) ;
#12555=VERTEX_POINT ( 'NONE', #46152 ) ;
#12556=DIRECTION ( 'NONE',  ( -0.000000000000000000, -1.000000000000000000, -0.000000000000000000 ) ) ;
#12557=ORIENTED_EDGE ( 'NONE', *, *, #119905, .F. ) ;
#12558=DIRECTION ( 'NONE',  ( -0.000000000000000000, -1.000000000000000000, -0.000000000000000000 ) ) ;
#12559=CARTESIAN_POINT ( 'NONE',  ( -8.350000000000012079, 12.50000000000000000, 2.857883832488649301 ) ) ;
#12560=EDGE_CURVE ( 'NONE', #48060, #115619, #93550, .T. ) ;
#12561=DIRECTION ( 'NONE',  ( 0.000000000000000000, -0.000000000000000000, 1.000000000000000000 ) ) ;
#12562=VERTEX_POINT ( 'NONE', #45526 ) ;
#12563=ORIENTED_EDGE ( 'NONE', *, *, #80438, .T. ) ;
#12564=FACE_BOUND ( 'NONE', #64909, .T. ) ;
#12565=ORIENTED_EDGE ( 'NONE', *, *, #96526, .T. ) ;
#12566=EDGE_CURVE ( 'NONE', #4284, #52488, #54667, .T. ) ;
#12567=CARTESIAN_POINT ( 'NONE',  ( -12.89999999999999147, 2.500000000000000000, 3.637306695894644726 ) ) ;
#12568=DIRECTION ( 'NONE',  ( 0.000000000000000000, 1.000000000000000000, 0.000000000000000000 ) ) ;
#12569=AXIS2_PLACEMENT_3D ( 'NONE', #20249, #42484, #60191 ) ;
#12570=DIRECTION ( 'NONE',  ( 0.000000000000000000, 0.000000000000000000, -1.000000000000000000 ) ) ;
#12571=DIRECTION ( 'NONE',  ( 0.000000000000000000, 0.000000000000000000, 1.000000000000000000 ) ) ;
#12572=CARTESIAN_POINT ( 'NONE',  ( -7.500000000000016875, 12.50000000000000000, -3.637306695894650055 ) ) ;
#12573=FACE_OUTER_BOUND ( 'NONE', #35219, .T. ) ;
#12574=DIRECTION ( 'NONE',  ( -0.000000000000000000, -1.000000000000000000, -0.000000000000000000 ) ) ;
#12575=CARTESIAN_POINT ( 'NONE',  ( -8.750000000000010658, 2.500000000000000000, -1.472243186433550122 ) ) ;
#12576=EDGE_CURVE ( 'NONE', #110135, #80892, #47592, .T. ) ;
#12577=DIRECTION ( 'NONE',  ( 0.000000000000000000, 0.000000000000000000, 1.000000000000000000 ) ) ;
#12578=CARTESIAN_POINT ( 'NONE',  ( -7.500000000000013323, 2.500000000000000000, 5.122947341949749323 ) ) ;
#12579=AXIS2_PLACEMENT_3D ( 'NONE', #99344, #39154, #88869 ) ;
#12580=DIRECTION ( 'NONE',  ( 0.000000000000000000, -0.9999939076577903929, 0.003490651415223739937 ) ) ;
#12581=AXIS2_PLACEMENT_3D ( 'NONE', #92347, #112011, #62271 ) ;
#12582=ORIENTED_EDGE ( 'NONE', *, *, #113846, .F. ) ;
#12584=VERTEX_POINT ( 'NONE', #115520 ) ;
#12585=CARTESIAN_POINT ( 'NONE',  ( -6.650000000000019007, 2.500000000000000000, -1.472243186433550122 ) ) ;
#12586=VERTEX_POINT ( 'NONE', #65787 ) ;
#12587=FACE_OUTER_BOUND ( 'NONE', #29336, .T. ) ;
#12588=CARTESIAN_POINT ( 'NONE',  ( -7.499999999999980460, 2.500000000000000000, 0.09999999999999772959 ) ) ;
#12589=ORIENTED_EDGE ( 'NONE', *, *, #123710, .T. ) ;
#12590=ORIENTED_EDGE ( 'NONE', *, *, #76516, .F. ) ;
#12591=EDGE_LOOP ( 'NONE', ( #122077, #90913, #107403, #35625 ) ) ;
#12592=PLANE ( 'NONE',  #33373 ) ;
#12593=AXIS2_PLACEMENT_3D ( 'NONE', #3213, #33956, #1902 ) ;
#12594=DIRECTION ( 'NONE',  ( 0.000000000000000000, -0.9999939076577903929, 0.003490651415223739937 ) ) ;
#12595=LINE ( 'NONE', #53196, #101488 ) ;
#12596=CIRCLE ( 'NONE', #73164, 0.06509327318403745899 ) ;
#12597=CARTESIAN_POINT ( 'NONE',  ( 8.149999999999923972, 12.50000000000000000, 2.511473670974873507 ) ) ;
#12598=DIRECTION ( 'NONE',  ( -4.274815082592931898E-19, -0.9999939076577903929, -0.003490651415223739937 ) ) ;
#12599=EDGE_LOOP ( 'NONE', ( #114201, #78716 ) ) ;
#12600=DIRECTION ( 'NONE',  ( 0.000000000000000000, 0.000000000000000000, 1.000000000000000000 ) ) ;
#12601=EDGE_LOOP ( 'NONE', ( #17738, #126446, #42075, #104591 ) ) ;
#12602=ADVANCED_FACE ( 'NONE', ( #16034 ), #66353, .T. ) ;
#12603=ORIENTED_EDGE ( 'NONE', *, *, #36725, .F. ) ;
#12604=ORIENTED_EDGE ( 'NONE', *, *, #18645, .F. ) ;
#12605=FACE_OUTER_BOUND ( 'NONE', #32055, .T. ) ;
#12606=EDGE_CURVE ( 'NONE', #120101, #31773, #120737, .T. ) ;
#12607=VERTEX_POINT ( 'NONE', #86726 ) ;
#12608=EDGE_CURVE ( 'NONE', #109560, #93720, #97749, .T. ) ;
#12609=ORIENTED_EDGE ( 'NONE', *, *, #21342, .F. ) ;
#12610=ADVANCED_FACE ( 'NONE', ( #93973 ), #9927, .T. ) ;
#12611=ORIENTED_EDGE ( 'NONE', *, *, #43262, .T. ) ;
#12612=ADVANCED_FACE ( 'NONE', ( #64504 ), #18324, .T. ) ;
#12615=DIRECTION ( 'NONE',  ( -0.000000000000000000, 1.000000000000000000, -0.000000000000000000 ) ) ;
#12616=DIRECTION ( 'NONE',  ( 0.000000000000000000, 0.000000000000000000, -1.000000000000000000 ) ) ;
#12617=PLANE ( 'NONE',  #90910 ) ;
#12618=EDGE_CURVE ( 'NONE', #27779, #81003, #51795, .T. ) ;
#12619=VECTOR ( 'NONE', #5523, 1000.000000000000000 ) ;
#12620=DIRECTION ( 'NONE',  ( -0.000000000000000000, -1.000000000000000000, -0.000000000000000000 ) ) ;
#12621=CONICAL_SURFACE ( 'NONE', #100458, 0.1000000000000000472, 0.003490658503988666988 ) ;
#12622=EDGE_CURVE ( 'NONE', #123263, #87808, #99821, .T. ) ;
#12623=LINE ( 'NONE', #11346, #74190 ) ;
#12624=VERTEX_POINT ( 'NONE', #27798 ) ;
#12625=CARTESIAN_POINT ( 'NONE',  ( 11.04999999999991189, 12.50000000000000000, 6.148780366869520897 ) ) ;
#12626=CIRCLE ( 'NONE', #83658, 0.1000000000000002554 ) ;
#12627=EDGE_CURVE ( 'NONE', #74873, #119487, #30879, .T. ) ;
#12628=ORIENTED_EDGE ( 'NONE', *, *, #95906, .T. ) ;
#12629=DIRECTION ( 'NONE',  ( 0.000000000000000000, 0.000000000000000000, 1.000000000000000000 ) ) ;
#12630=ORIENTED_EDGE ( 'NONE', *, *, #60865, .T. ) ;
#12631=CARTESIAN_POINT ( 'NONE',  ( -14.54999999999998472, 2.500000000000000000, -2.165063509461099489 ) ) ;
#12632=EDGE_CURVE ( 'NONE', #24019, #90957, #76833, .T. ) ;
#12633=VERTEX_POINT ( 'NONE', #78865 ) ;
#12634=ADVANCED_FACE ( 'NONE', ( #116822 ), #58571, .T. ) ;
#12636=FACE_OUTER_BOUND ( 'NONE', #43915, .T. ) ;
#12638=ORIENTED_EDGE ( 'NONE', *, *, #81778, .T. ) ;
#12639=FACE_OUTER_BOUND ( 'NONE', #72557, .T. ) ;
#12641=DIRECTION ( 'NONE',  ( -0.000000000000000000, -1.000000000000000000, -0.000000000000000000 ) ) ;
#12642=DIRECTION ( 'NONE',  ( 0.000000000000000000, 0.000000000000000000, 1.000000000000000000 ) ) ;
#12643=DIRECTION ( 'NONE',  ( 0.000000000000000000, -0.9999939076577903929, 0.003490651415223739937 ) ) ;
#12644=VERTEX_POINT ( 'NONE', #48099 ) ;
#12645=FACE_OUTER_BOUND ( 'NONE', #50166, .T. ) ;
#12646=EDGE_LOOP ( 'NONE', ( #63428, #126757 ) ) ;
#12648=AXIS2_PLACEMENT_3D ( 'NONE', #46610, #49217, #38760 ) ;
#12649=CARTESIAN_POINT ( 'NONE',  ( 16.56576425165007649, 1.499999999999997113, 6.084390597445792359 ) ) ;
#12650=AXIS2_PLACEMENT_3D ( 'NONE', #92812, #122270, #104549 ) ;
#12652=CARTESIAN_POINT ( 'NONE',  ( -12.29999999999999361, 2.500000000000000000, 3.983716857408420076 ) ) ;
#12653=CARTESIAN_POINT ( 'NONE',  ( 6.649999999999930189, 2.500000000000000000, 7.188010851410848723 ) ) ;
#12654=LINE ( 'NONE', #53252, #20950 ) ;
#12655=DIRECTION ( 'NONE',  ( -0.000000000000000000, -1.000000000000000000, -0.000000000000000000 ) ) ;
#12656=ORIENTED_EDGE ( 'NONE', *, *, #47476, .T. ) ;
#12657=AXIS2_PLACEMENT_3D ( 'NONE', #107171, #78386, #27979 ) ;
#12658=CARTESIAN_POINT ( 'NONE',  ( -1.850000000000033396, 2.500000000000000000, -6.841600689897077814 ) ) ;
#12659=EDGE_CURVE ( 'NONE', #45310, #24791, #39203, .T. ) ;
#12660=DIRECTION ( 'NONE',  ( -0.000000000000000000, -1.000000000000000000, -0.000000000000000000 ) ) ;
#12661=DIRECTION ( 'NONE',  ( -0.000000000000000000, -1.000000000000000000, -0.000000000000000000 ) ) ;
#12662=ADVANCED_FACE ( 'NONE', ( #38284 ), #24592, .T. ) ;
#12663=ORIENTED_EDGE ( 'NONE', *, *, #115691, .T. ) ;
#12664=EDGE_LOOP ( 'NONE', ( #124265, #118232, #71065, #28463 ) ) ;
#12665=DIRECTION ( 'NONE',  ( 0.000000000000000000, 0.000000000000000000, 1.000000000000000000 ) ) ;
#12666=CIRCLE ( 'NONE', #39896, 0.06509327318403745899 ) ;
#12667=CONICAL_SURFACE ( 'NONE', #127614, 0.1000000000000000472, 0.003490658503988666988 ) ;
#12668=EDGE_LOOP ( 'NONE', ( #52401, #60273, #102475, #108856 ) ) ;
#12669=PRODUCT_DEFINITION_SHAPE ( 'NONE', 'NONE',  #65974 ) ;
#12670=ORIENTED_EDGE ( 'NONE', *, *, #12766, .T. ) ;
#12672=EDGE_LOOP ( 'NONE', ( #117271, #36574, #59509, #77487 ) ) ;
#12673=CARTESIAN_POINT ( 'NONE',  ( 20.69433222467976208, -2.585316282074205496, -4.139109617397429552 ) ) ;
#12674=DIRECTION ( 'NONE',  ( 0.000000000000000000, 0.000000000000000000, 1.000000000000000000 ) ) ;
#12675=CARTESIAN_POINT ( 'NONE',  ( 19.51231976789225797, 0.5900868802304030103, 4.348342248683020550 ) ) ;
#12676=AXIS2_PLACEMENT_3D ( 'NONE', #58750, #48938, #109110 ) ;
#12677=ORIENTED_EDGE ( 'NONE', *, *, #99262, .T. ) ;
#12678=CARTESIAN_POINT ( 'NONE',  ( -10.20000000000000462, 12.50000000000000000, 4.611443907251934426 ) ) ;
#12679=CARTESIAN_POINT ( 'NONE',  ( 15.79999999999989058, 12.50000000000000000, 0.06509327318403504425 ) ) ;
#12680=VECTOR ( 'NONE', #8202, 1000.000000000000000 ) ;
#12683=EDGE_LOOP ( 'NONE', ( #12019, #62559 ) ) ;
#12684=LINE ( 'NONE', #120725, #56668 ) ;
#12685=CARTESIAN_POINT ( 'NONE',  ( 3.349999999999941025, 12.50000000000000000, 7.188010851410848723 ) ) ;
#12686=DIRECTION ( 'NONE',  ( 0.000000000000000000, 1.000000000000000000, 0.000000000000000000 ) ) ;
#12687=FACE_BOUND ( 'NONE', #5639, .T. ) ;
#12688=ORIENTED_EDGE ( 'NONE', *, *, #99674, .F. ) ;
#12689=CARTESIAN_POINT ( 'NONE',  ( 8.949999999999921130, 2.500000000000000000, 1.818653347947321475 ) ) ;
#12690=DIRECTION ( 'NONE',  ( -0.000000000000000000, 1.000000000000000000, -0.000000000000000000 ) ) ;
#12691=EDGE_LOOP ( 'NONE', ( #88494, #5179 ) ) ;
#12692=DIRECTION ( 'NONE',  ( 0.000000000000000000, -0.9999939076577903929, 0.003490651415223739937 ) ) ;
#12693=ADVANCED_FACE ( 'NONE', ( #27161 ), #99135, .T. ) ;
#12694=DIRECTION ( 'NONE',  ( 0.000000000000000000, 0.000000000000000000, 1.000000000000000000 ) ) ;
#12696=CARTESIAN_POINT ( 'NONE',  ( -3.150000000000029221, 12.50000000000000000, -1.818653347947326138 ) ) ;
#12697=FACE_OUTER_BOUND ( 'NONE', #51202, .T. ) ;
#12698=DIRECTION ( 'NONE',  ( 0.000000000000000000, 1.000000000000000000, 0.000000000000000000 ) ) ;
#12699=AXIS2_PLACEMENT_3D ( 'NONE', #42778, #93145, #81398 ) ;
#12700=CONICAL_SURFACE ( 'NONE', #48231, 0.1000000000000002554, 0.003490658503988666988 ) ;
#12701=CARTESIAN_POINT ( 'NONE',  ( -3.300000000000028244, 2.500000000000000000, 4.330127018922196314 ) ) ;
#12702=DIRECTION ( 'NONE',  ( 0.000000000000000000, 0.000000000000000000, 1.000000000000000000 ) ) ;
#12703=EDGE_CURVE ( 'NONE', #124476, #84951, #106071, .T. ) ;
#12704=CONICAL_SURFACE ( 'NONE', #100461, 0.1000000000000000056, 0.003490658503988666988 ) ;
#12705=EDGE_LOOP ( 'NONE', ( #84564, #71154, #60604 ) ) ;
#12706=VERTEX_POINT ( 'NONE', #19933 ) ;
#12707=ORIENTED_EDGE ( 'NONE', *, *, #18228, .F. ) ;
#12708=VERTEX_POINT ( 'NONE', #127943 ) ;
#12709=CARTESIAN_POINT ( 'NONE',  ( -13.54999999999999005, 12.50000000000000000, -1.818653347947323917 ) ) ;
#12710=CARTESIAN_POINT ( 'NONE',  ( -6.450000000000017941, 2.500000000000000000, -6.841600689897077814 ) ) ;
#12711=CONICAL_SURFACE ( 'NONE', #46177, 0.1000000000000002554, 0.003490658503988666988 ) ;
#12712=EDGE_CURVE ( 'NONE', #25509, #122967, #41343, .T. ) ;
#12713=DIRECTION ( 'NONE',  ( -0.000000000000000000, 1.000000000000000000, -0.000000000000000000 ) ) ;
#12715=FACE_BOUND ( 'NONE', #1588, .T. ) ;
#12716=EDGE_CURVE ( 'NONE', #105608, #43127, #70560, .T. ) ;
#12717=CARTESIAN_POINT ( 'NONE',  ( -1.850000000000033396, 12.50000000000000000, -6.148780366869526226 ) ) ;
#12718=DIRECTION ( 'NONE',  ( 0.000000000000000000, 1.000000000000000000, 0.000000000000000000 ) ) ;
#12719=LINE ( 'NONE', #112234, #105599 ) ;
#12720=CARTESIAN_POINT ( 'NONE',  ( 11.64999999999990443, 12.50000000000000000, -7.188010851410854052 ) ) ;
#12721=CARTESIAN_POINT ( 'NONE',  ( 7.099999999999925926, 12.50000000000000000, 0.6277270498435120194 ) ) ;
#12723=CARTESIAN_POINT ( 'NONE',  ( 12.49999999999990408, 2.500000000000000000, -3.537306695894649966 ) ) ;
#12724=FACE_OUTER_BOUND ( 'NONE', #8167, .T. ) ;
#12725=EDGE_CURVE ( 'NONE', #119819, #19084, #68370, .T. ) ;
#12726=CARTESIAN_POINT ( 'NONE',  ( 6.249999999999930722, 2.500000000000000000, 1.472243186433545459 ) ) ;
#12727=ORIENTED_EDGE ( 'NONE', *, *, #101038, .F. ) ;
#12728=AXIS2_PLACEMENT_3D ( 'NONE', #56842, #47061, #126255 ) ;
#12729=ORIENTED_EDGE ( 'NONE', *, *, #24437, .F. ) ;
#12730=EDGE_LOOP ( 'NONE', ( #55631, #86431, #69249, #56418 ) ) ;
#12731=ORIENTED_EDGE ( 'NONE', *, *, #124485, .F. ) ;
#12732=ORIENTED_EDGE ( 'NONE', *, *, #82404, .T. ) ;
#12734=LINE ( 'NONE', #40291, #94467 ) ;
#12735=ORIENTED_EDGE ( 'NONE', *, *, #106988, .F. ) ;
#12736=VERTEX_POINT ( 'NONE', #57272 ) ;
#12737=VECTOR ( 'NONE', #111155, 1000.000000000000000 ) ;
#12738=AXIS2_PLACEMENT_3D ( 'NONE', #52712, #92640, #3616 ) ;
#12739=FACE_OUTER_BOUND ( 'NONE', #110728, .T. ) ;
#12740=DIRECTION ( 'NONE',  ( 0.000000000000000000, -0.9999939076577903929, 0.003490651415223739937 ) ) ;
#12741=DIRECTION ( 'NONE',  ( -4.274815082592931898E-19, -0.9999939076577903929, -0.003490651415223739937 ) ) ;
#12742=ORIENTED_EDGE ( 'NONE', *, *, #120350, .F. ) ;
#12743=DIRECTION ( 'NONE',  ( -0.000000000000000000, 1.000000000000000000, -0.000000000000000000 ) ) ;
#12744=AXIS2_PLACEMENT_3D ( 'NONE', #26849, #96866, #55659 ) ;
#12745=CIRCLE ( 'NONE', #31551, 0.06509327318403745899 ) ;
#12746=EDGE_LOOP ( 'NONE', ( #65342, #85770, #82161, #94063 ) ) ;
#12747=ADVANCED_FACE ( 'NONE', ( #91244 ), #42144, .T. ) ;
#12748=VERTEX_POINT ( 'NONE', #32985 ) ;
#12749=CARTESIAN_POINT ( 'NONE',  ( 3.149999999999942624, 2.500000000000000000, 6.841600689897072485 ) ) ;
#12750=DIRECTION ( 'NONE',  ( 0.000000000000000000, 0.000000000000000000, 1.000000000000000000 ) ) ;
#12751=EDGE_CURVE ( 'NONE', #121932, #20597, #122794, .T. ) ;
#12753=ORIENTED_EDGE ( 'NONE', *, *, #98019, .F. ) ;
#12754=EDGE_CURVE ( 'NONE', #100839, #47341, #43398, .T. ) ;
#12755=AXIS2_PLACEMENT_3D ( 'NONE', #37951, #100101, #89633 ) ;
#12756=DIRECTION ( 'NONE',  ( 0.000000000000000000, 0.000000000000000000, 1.000000000000000000 ) ) ;
#12757=AXIS2_PLACEMENT_3D ( 'NONE', #43001, #122821, #99961 ) ;
#12758=DIRECTION ( 'NONE',  ( -0.000000000000000000, -1.000000000000000000, -0.000000000000000000 ) ) ;
#12759=CARTESIAN_POINT ( 'NONE',  ( 1.699999999999951994, 2.500000000000000000, 0.09999999999999772959 ) ) ;
#12760=FACE_OUTER_BOUND ( 'NONE', #48640, .T. ) ;
#12761=EDGE_CURVE ( 'NONE', #89951, #37339, #116524, .T. ) ;
#12762=EDGE_CURVE ( 'NONE', #55354, #16720, #110863, .T. ) ;
#12763=FACE_OUTER_BOUND ( 'NONE', #102474, .T. ) ;
#12764=ADVANCED_FACE ( 'NONE', ( #72894 ), #60514, .T. ) ;
#12765=CONICAL_SURFACE ( 'NONE', #71353, 0.1000000000000002554, 0.003490658503988666988 ) ;
#12766=EDGE_CURVE ( 'NONE', #17565, #88843, #108213, .T. ) ;
#12767=EDGE_LOOP ( 'NONE', ( #26867, #5617, #30942, #60544 ) ) ;
#12768=CARTESIAN_POINT ( 'NONE',  ( 4.849235612580096166, -2.499999999999999112, 8.943930330244963756 ) ) ;
#12769=EDGE_LOOP ( 'NONE', ( #108321, #96886 ) ) ;
#12770=DIRECTION ( 'NONE',  ( -4.274815082592931898E-19, -0.9999939076577903929, -0.003490651415223739937 ) ) ;
#12771=ADVANCED_FACE ( 'NONE', ( #10718 ), #82731, .T. ) ;
#12772=CARTESIAN_POINT ( 'NONE',  ( 6.249999999999967137, 2.500000000000000000, -2.165063509461101710 ) ) ;
#12773=AXIS2_PLACEMENT_3D ( 'NONE', #78262, #99829, #10150 ) ;
#12774=AXIS2_PLACEMENT_3D ( 'NONE', #68485, #7623, #126120 ) ;
#12775=FACE_OUTER_BOUND ( 'NONE', #20598, .T. ) ;
#12776=LINE ( 'NONE', #61913, #38291 ) ;
#12777=PLANE ( 'NONE',  #123298 ) ;
#12778=ORIENTED_EDGE ( 'NONE', *, *, #123318, .F. ) ;
#12779=ADVANCED_FACE ( 'NONE', ( #52598 ), #7954, .T. ) ;
#12780=PLANE ( 'NONE',  #46783 ) ;
#12781=FACE_OUTER_BOUND ( 'NONE', #12591, .T. ) ;
#12782=ORIENTED_EDGE ( 'NONE', *, *, #6397, .F. ) ;
#12783=EDGE_LOOP ( 'NONE', ( #31804, #120980 ) ) ;
#12784=ORIENTED_EDGE ( 'NONE', *, *, #11639, .T. ) ;
#12785=CARTESIAN_POINT ( 'NONE',  ( -13.09999999999999254, 2.500000000000000000, -4.676537180435975216 ) ) ;
#12786=DIRECTION ( 'NONE',  ( 0.000000000000000000, -0.000000000000000000, 1.000000000000000000 ) ) ;
#12788=LINE ( 'NONE', #101837, #107627 ) ;
#12789=LINE ( 'NONE', #92661, #11032 ) ;
#12790=CARTESIAN_POINT ( 'NONE',  ( 5.449999999999937117, 2.500000000000000000, -6.495190528383302464 ) ) ;
#12792=AXIS2_PLACEMENT_3D ( 'NONE', #124365, #71369, #53685 ) ;
#12793=AXIS2_PLACEMENT_3D ( 'NONE', #7964, #49849, #39398 ) ;
#12794=AXIS2_PLACEMENT_3D ( 'NONE', #72844, #92474, #82010 ) ;
#12795=CARTESIAN_POINT ( 'NONE',  ( 4.599999999999939249, 2.500000000000000000, -3.737306695894649700 ) ) ;
#12796=AXIS2_PLACEMENT_3D ( 'NONE', #97278, #7601, #108386 ) ;
#12797=ORIENTED_EDGE ( 'NONE', *, *, #10165, .T. ) ;
#12798=PLANE ( 'NONE',  #8817 ) ;
#12799=CIRCLE ( 'NONE', #75504, 0.1000000000000000472 ) ;
#12800=DIRECTION ( 'NONE',  ( 0.000000000000000000, 0.000000000000000000, 1.000000000000000000 ) ) ;
#12802=DIRECTION ( 'NONE',  ( -0.000000000000000000, 1.000000000000000000, -0.000000000000000000 ) ) ;
#12803=ORIENTED_EDGE ( 'NONE', *, *, #47964, .T. ) ;
#12804=DIRECTION ( 'NONE',  ( 0.000000000000000000, 0.000000000000000000, 1.000000000000000000 ) ) ;
#12805=EDGE_CURVE ( 'NONE', #72699, #78169, #66441, .T. ) ;
#12806=FACE_OUTER_BOUND ( 'NONE', #8709, .T. ) ;
#12807=DIRECTION ( 'NONE',  ( -4.274815082592931898E-19, -0.9999939076577903929, -0.003490651415223739937 ) ) ;
#12808=ORIENTED_EDGE ( 'NONE', *, *, #72062, .T. ) ;
#12809=ORIENTED_EDGE ( 'NONE', *, *, #110170, .T. ) ;
#12810=CARTESIAN_POINT ( 'NONE',  ( -6.050000000000018474, 2.500000000000000000, 2.411473670974873862 ) ) ;
#12811=EDGE_CURVE ( 'NONE', #71464, #106656, #72718, .T. ) ;
#12812=EDGE_LOOP ( 'NONE', ( #95821, #61386 ) ) ;
#12813=EDGE_LOOP ( 'NONE', ( #69645, #114652, #16410, #104519 ) ) ;
#12814=CARTESIAN_POINT ( 'NONE',  ( -9.350000000000008527, 2.500000000000000000, -6.248780366869521430 ) ) ;
#12815=CARTESIAN_POINT ( 'NONE',  ( 16.09541403888750821, 2.463474929527661228, -3.723514363709292230 ) ) ;
#12816=FACE_OUTER_BOUND ( 'NONE', #96765, .T. ) ;
#12817=DIRECTION ( 'NONE',  ( 0.000000000000000000, 0.000000000000000000, -1.000000000000000000 ) ) ;
#12818=AXIS2_PLACEMENT_3D ( 'NONE', #44367, #54825, #115031 ) ;
#12819=ORIENTED_EDGE ( 'NONE', *, *, #71286, .F. ) ;
#12820=AXIS2_PLACEMENT_3D ( 'NONE', #107617, #86015, #45491 ) ;
#12821=DIRECTION ( 'NONE',  ( -0.000000000000000000, 1.000000000000000000, -0.000000000000000000 ) ) ;
#12822=CARTESIAN_POINT ( 'NONE',  ( -2.500000000000032419, 2.500000000000000000, -3.637306695894650055 ) ) ;
#12823=VERTEX_POINT ( 'NONE', #101061 ) ;
#12824=DIRECTION ( 'NONE',  ( -4.274815082592931898E-19, -0.9999939076577903929, -0.003490651415223739937 ) ) ;
#12825=CARTESIAN_POINT ( 'NONE',  ( -15.39999999999997904, 12.50000000000000000, 0.000000000000000000 ) ) ;
#12826=CONICAL_SURFACE ( 'NONE', #77684, 0.1000000000000002554, 0.003490658503988666988 ) ;
#12827=EDGE_LOOP ( 'NONE', ( #110677, #52022, #29077, #115494 ) ) ;
#12829=ORIENTED_EDGE ( 'NONE', *, *, #111132, .F. ) ;
#12830=ORIENTED_EDGE ( 'NONE', *, *, #113883, .F. ) ;
#12831=VERTEX_POINT ( 'NONE', #31678 ) ;
#12832=DIRECTION ( 'NONE',  ( 0.000000000000000000, 0.000000000000000000, 1.000000000000000000 ) ) ;
#12833=CARTESIAN_POINT ( 'NONE',  ( 12.65326442544382601, 1.500000000000126121, 8.428886915957018999 ) ) ;
#12834=DIRECTION ( 'NONE',  ( 0.000000000000000000, 1.000000000000000000, 0.000000000000000000 ) ) ;
#12835=FACE_BOUND ( 'NONE', #75695, .T. ) ;
#12836=ORIENTED_EDGE ( 'NONE', *, *, #55600, .F. ) ;
#12838=DIRECTION ( 'NONE',  ( -1.000000000000000000, 0.000000000000000000, 0.000000000000000000 ) ) ;
#12839=DIRECTION ( 'NONE',  ( 0.000000000000000000, 0.000000000000000000, -1.000000000000000000 ) ) ;
#12840=CIRCLE ( 'NONE', #94326, 0.06509327318403745899 ) ;
#12842=CONICAL_SURFACE ( 'NONE', #92277, 0.1000000000000002554, 0.003490658503988666988 ) ;
#12843=EDGE_CURVE ( 'NONE', #105744, #89132, #83192, .T. ) ;
#12844=CIRCLE ( 'NONE', #127795, 0.1000000000000000056 ) ;
#12845=DIRECTION ( 'NONE',  ( 0.000000000000000000, 0.000000000000000000, 1.000000000000000000 ) ) ;
#12846=CARTESIAN_POINT ( 'NONE',  ( 0.5999999999999612310, 12.50000000000000000, -0.3464101615137760715 ) ) ;
#12847=CARTESIAN_POINT ( 'NONE',  ( 11.69999999999990870, 2.500000000000000000, -4.230127018922201998 ) ) ;
#12848=AXIS2_PLACEMENT_3D ( 'NONE', #38986, #38314, #99166 ) ;
#12849=EDGE_CURVE ( 'NONE', #4351, #91437, #92523, .T. ) ;
#12850=PLANE ( 'NONE',  #93429 ) ;
#12851=ORIENTED_EDGE ( 'NONE', *, *, #54688, .F. ) ;
#12852=VECTOR ( 'NONE', #41404, 1000.000000000000000 ) ;
#12853=VECTOR ( 'NONE', #105024, 1000.000000000000000 ) ;
#12854=ORIENTED_EDGE ( 'NONE', *, *, #121851, .T. ) ;
#12855=EDGE_LOOP ( 'NONE', ( #101725, #13205 ) ) ;
#12856=ORIENTED_EDGE ( 'NONE', *, *, #74995, .F. ) ;
#12858=DIRECTION ( 'NONE',  ( 0.000000000000000000, -0.000000000000000000, 1.000000000000000000 ) ) ;
#12859=ADVANCED_FACE ( 'NONE', ( #121338 ), #12067, .T. ) ;
#12860=DIRECTION ( 'NONE',  ( 0.000000000000000000, 1.000000000000000000, 0.000000000000000000 ) ) ;
#12861=EDGE_LOOP ( 'NONE', ( #129108, #27964, #53069, #114743 ) ) ;
#12862=FACE_BOUND ( 'NONE', #26514, .T. ) ;
#12863=EDGE_CURVE ( 'NONE', #60734, #50580, #3756, .T. ) ;
#12864=CARTESIAN_POINT ( 'NONE',  ( 12.04999999999990834, 2.500000000000000000, 6.495190528383297135 ) ) ;
#12865=EDGE_CURVE ( 'NONE', #124, #100363, #14205, .T. ) ;
#12866=ORIENTED_EDGE ( 'NONE', *, *, #122875, .T. ) ;
#12867=CARTESIAN_POINT ( 'NONE',  ( -4.200000000000025935, 12.50000000000000000, -0.06509327318403980434 ) ) ;
#12868=DIRECTION ( 'NONE',  ( 0.000000000000000000, 0.000000000000000000, -1.000000000000000000 ) ) ;
#12869=EDGE_CURVE ( 'NONE', #7967, #81575, #104108, .T. ) ;
#12870=DIRECTION ( 'NONE',  ( 0.000000000000000000, 0.000000000000000000, -1.000000000000000000 ) ) ;
#12871=EDGE_LOOP ( 'NONE', ( #119711, #42935 ) ) ;
#12872=PLANE ( 'NONE',  #7414 ) ;
#12873=ORIENTED_EDGE ( 'NONE', *, *, #21395, .F. ) ;
#12874=ORIENTED_EDGE ( 'NONE', *, *, #58870, .F. ) ;
#12875=CIRCLE ( 'NONE', #4550, 0.06509327318403745899 ) ;
#12877=AXIS2_PLACEMENT_3D ( 'NONE', #57410, #127444, #117584 ) ;
#12878=DIRECTION ( 'NONE',  ( -0.000000000000000000, 1.000000000000000000, -0.000000000000000000 ) ) ;
#12879=DIRECTION ( 'NONE',  ( 0.000000000000000000, 1.000000000000000000, 0.000000000000000000 ) ) ;
#12880=DIRECTION ( 'NONE',  ( 0.000000000000000000, 0.000000000000000000, -1.000000000000000000 ) ) ;
#12881=ORIENTED_EDGE ( 'NONE', *, *, #30183, .T. ) ;
#12882=DIRECTION ( 'NONE',  ( 0.000000000000000000, 0.000000000000000000, 1.000000000000000000 ) ) ;
#12883=CARTESIAN_POINT ( 'NONE',  ( -1.250000000000001554, 2.500000000000000000, 2.265063509461097357 ) ) ;
#12884=AXIS2_PLACEMENT_3D ( 'NONE', #25388, #16206, #37176 ) ;
#12885=AXIS2_PLACEMENT_3D ( 'NONE', #50765, #42239, #62530 ) ;
#12886=CARTESIAN_POINT ( 'NONE',  ( 3.149999999999944400, 12.50000000000000000, 2.446380397790835826 ) ) ;
#12888=ORIENTED_EDGE ( 'NONE', *, *, #52411, .F. ) ;
#12889=AXIS2_PLACEMENT_3D ( 'NONE', #10183, #50121, #122076 ) ;
#12890=AXIS2_PLACEMENT_3D ( 'NONE', #73520, #71598, #21872 ) ;
#12891=DIRECTION ( 'NONE',  ( 0.000000000000000000, 0.000000000000000000, 1.000000000000000000 ) ) ;
#12892=ORIENTED_EDGE ( 'NONE', *, *, #12042, .F. ) ;
#12893=DIRECTION ( 'NONE',  ( 0.000000000000000000, 1.000000000000000000, 0.000000000000000000 ) ) ;
#12894=AXIS2_PLACEMENT_3D ( 'NONE', #33812, #66485, #113665 ) ;
#12895=EDGE_LOOP ( 'NONE', ( #49454, #17572 ) ) ;
#12896=EDGE_LOOP ( 'NONE', ( #62833, #995, #126214, #11628 ) ) ;
#12897=FACE_OUTER_BOUND ( 'NONE', #69951, .T. ) ;
#12898=DIRECTION ( 'NONE',  ( 0.000000000000000000, 0.000000000000000000, 1.000000000000000000 ) ) ;
#12899=DIRECTION ( 'NONE',  ( 0.000000000000000000, 1.000000000000000000, 0.000000000000000000 ) ) ;
#12900=LINE ( 'NONE', #41122, #94755 ) ;
#12901=DIRECTION ( 'NONE',  ( 0.000000000000000000, -0.9999939076577903929, 0.003490651415223739937 ) ) ;
#12902=VERTEX_POINT ( 'NONE', #101716 ) ;
#12903=EDGE_LOOP ( 'NONE', ( #66424, #33366 ) ) ;
#12904=DIRECTION ( 'NONE',  ( -4.274815082592931898E-19, -0.9999939076577903929, -0.003490651415223739937 ) ) ;
#12905=CARTESIAN_POINT ( 'NONE',  ( 11.84999999999990372, 2.500000000000000000, 2.511473670974873507 ) ) ;
#12906=PLANE ( 'NONE',  #87735 ) ;
#12907=EDGE_CURVE ( 'NONE', #37067, #11332, #75457, .T. ) ;
#12908=ORIENTED_EDGE ( 'NONE', *, *, #10704, .T. ) ;
#12909=ORIENTED_EDGE ( 'NONE', *, *, #30355, .F. ) ;
#12910=EDGE_CURVE ( 'NONE', #6482, #86589, #41437, .T. ) ;
#12911=FACE_OUTER_BOUND ( 'NONE', #106112, .T. ) ;
#12912=EDGE_CURVE ( 'NONE', #52516, #99205, #62265, .T. ) ;
#12914=CIRCLE ( 'NONE', #115398, 0.1000000000000000472 ) ;
#12915=ORIENTED_EDGE ( 'NONE', *, *, #37051, .T. ) ;
#12916=DIRECTION ( 'NONE',  ( -0.000000000000000000, 1.000000000000000000, -0.000000000000000000 ) ) ;
#12917=DIRECTION ( 'NONE',  ( -0.000000000000000000, -1.000000000000000000, -0.000000000000000000 ) ) ;
#12918=CIRCLE ( 'NONE', #61056, 0.06509327318403745899 ) ;
#12919=CARTESIAN_POINT ( 'NONE',  ( -1.850000000000033840, 2.500000000000000000, 6.148780366869520897 ) ) ;
#12920=EDGE_LOOP ( 'NONE', ( #64529, #47148 ) ) ;
#12921=FACE_OUTER_BOUND ( 'NONE', #770, .T. ) ;
#12922=CARTESIAN_POINT ( 'NONE',  ( 8.299999999999922551, 12.50000000000000000, -2.385244779468109755E-15 ) ) ;
#12923=ADVANCED_FACE ( 'NONE', ( #85911 ), #43483, .T. ) ;
#12924=CARTESIAN_POINT ( 'NONE',  ( 3.149999999999946176, 12.50000000000000000, -6.083687093685488989 ) ) ;
#12925=DIRECTION ( 'NONE',  ( -0.000000000000000000, 1.000000000000000000, -0.000000000000000000 ) ) ;
#12927=CIRCLE ( 'NONE', #25442, 0.06509327318403745899 ) ;
#12928=ORIENTED_EDGE ( 'NONE', *, *, #33874, .F. ) ;
#12929=VECTOR ( 'NONE', #9411, 1000.000000000000000 ) ;
#12930=ADVANCED_FACE ( 'NONE', ( #14594 ), #30973, .T. ) ;
#12931=VECTOR ( 'NONE', #119865, 1000.000000000000000 ) ;
#12932=LINE ( 'NONE', #26007, #78065 ) ;
#12933=EDGE_CURVE ( 'NONE', #67119, #124524, #20493, .T. ) ;
#12934=AXIS2_PLACEMENT_3D ( 'NONE', #32492, #46630, #33125 ) ;
#12935=CARTESIAN_POINT ( 'NONE',  ( 48.83465639038744399, -3.619824997313607629, 4.313881469055892204 ) ) ;
#12936=ORIENTED_EDGE ( 'NONE', *, *, #86951, .T. ) ;
#12937=EDGE_LOOP ( 'NONE', ( #64563, #74537 ) ) ;
#12939=DIRECTION ( 'NONE',  ( 0.000000000000000000, 0.000000000000000000, 1.000000000000000000 ) ) ;
#12940=CARTESIAN_POINT ( 'NONE',  ( 8.349999999999919709, 2.500000000000000000, 6.495190528383297135 ) ) ;
#12941=AXIS2_PLACEMENT_3D ( 'NONE', #33767, #14745, #46168 ) ;
#12942=DIRECTION ( 'NONE',  ( -0.000000000000000000, -1.000000000000000000, -0.000000000000000000 ) ) ;
#12943=DIRECTION ( 'NONE',  ( -0.000000000000000000, 1.000000000000000000, -0.000000000000000000 ) ) ;
#12944=CIRCLE ( 'NONE', #25461, 0.06509327318403745899 ) ;
#12945=DIRECTION ( 'NONE',  ( -0.000000000000000000, 1.000000000000000000, -0.000000000000000000 ) ) ;
#12946=AXIS2_PLACEMENT_3D ( 'NONE', #61006, #19129, #119282 ) ;
#12947=FACE_OUTER_BOUND ( 'NONE', #57257, .T. ) ;
#12948=VECTOR ( 'NONE', #50605, 1000.000000000000000 ) ;
#12949=LINE ( 'NONE', #112472, #58235 ) ;
#12950=AXIS2_PLACEMENT_3D ( 'NONE', #106437, #118194, #128014 ) ;
#12951=FACE_OUTER_BOUND ( 'NONE', #108264, .T. ) ;
#12952=ORIENTED_EDGE ( 'NONE', *, *, #51164, .F. ) ;
#12953=ORIENTED_EDGE ( 'NONE', *, *, #96376, .T. ) ;
#12954=CONICAL_SURFACE ( 'NONE', #86107, 0.1000000000000002554, 0.003490658503988666988 ) ;
#12955=ORIENTED_EDGE ( 'NONE', *, *, #51806, .T. ) ;
#12956=ORIENTED_EDGE ( 'NONE', *, *, #83692, .F. ) ;
#12957=CARTESIAN_POINT ( 'NONE',  ( 4.549999999999937650, 2.500000000000000000, 2.165063509461097713 ) ) ;
#12959=VERTEX_POINT ( 'NONE', #85281 ) ;
#12960=DIRECTION ( 'NONE',  ( 0.000000000000000000, -0.000000000000000000, 1.000000000000000000 ) ) ;
#12961=FACE_OUTER_BOUND ( 'NONE', #119278, .T. ) ;
#12962=DIRECTION ( 'NONE',  ( -0.000000000000000000, 1.000000000000000000, -0.000000000000000000 ) ) ;
#12963=VERTEX_POINT ( 'NONE', #65639 ) ;
#12964=CARTESIAN_POINT ( 'NONE',  ( -6.450000000000014388, 2.500000000000000000, 6.148780366869520897 ) ) ;
#12965=DIRECTION ( 'NONE',  ( 0.000000000000000000, 0.000000000000000000, -1.000000000000000000 ) ) ;
#12966=EDGE_LOOP ( 'NONE', ( #18068, #57686 ) ) ;
#12968=EDGE_LOOP ( 'NONE', ( #71103, #30822, #115175, #19692 ) ) ;
#12969=VERTEX_POINT ( 'NONE', #15890 ) ;
#12970=VERTEX_POINT ( 'NONE', #45378 ) ;
#12971=CARTESIAN_POINT ( 'NONE',  ( -5.600000000000023626, 2.500000000000000000, -4.083716857408426826 ) ) ;
#12972=AXIS2_PLACEMENT_3D ( 'NONE', #68771, #79258, #60276 ) ;
#12973=CONICAL_SURFACE ( 'NONE', #48506, 0.09999999999999982514, 0.003490658503988666988 ) ;
#12974=DIRECTION ( 'NONE',  ( 0.000000000000000000, -0.9999939076577903929, 0.003490651415223739937 ) ) ;
#12976=CARTESIAN_POINT ( 'NONE',  ( -10.40000000000000213, 12.50000000000000000, 3.637306695894644726 ) ) ;
#12977=CIRCLE ( 'NONE', #44393, 0.09999999999999999167 ) ;
#12978=EDGE_LOOP ( 'NONE', ( #79196, #129369, #117893, #207 ) ) ;
#12979=AXIS2_PLACEMENT_3D ( 'NONE', #75917, #16960, #126317 ) ;
#12980=VECTOR ( 'NONE', #19031, 1000.000000000000000 ) ;
#12981=FACE_OUTER_BOUND ( 'NONE', #118782, .T. ) ;
#12982=AXIS2_PLACEMENT_3D ( 'NONE', #19172, #66991, #27093 ) ;
#12983=EDGE_LOOP ( 'NONE', ( #106410, #82037 ) ) ;
#12985=CARTESIAN_POINT ( 'NONE',  ( 4.912722231850287002, -2.499999999999493738, -9.942384338125227927 ) ) ;
#12986=CONICAL_SURFACE ( 'NONE', #67350, 0.09999999999999982514, 0.003490658503988666988 ) ;
#12987=DIRECTION ( 'NONE',  ( 0.000000000000000000, 0.000000000000000000, 1.000000000000000000 ) ) ;
#12988=FACE_OUTER_BOUND ( 'NONE', #71014, .T. ) ;
#12989=AXIS2_PLACEMENT_3D ( 'NONE', #3155, #51614, #122930 ) ;
#12990=ORIENTED_EDGE ( 'NONE', *, *, #66351, .F. ) ;
#12992=EDGE_LOOP ( 'NONE', ( #57182, #49158, #122128, #70930 ) ) ;
#12993=DIRECTION ( 'NONE',  ( 0.000000000000000000, 1.000000000000000000, 0.000000000000000000 ) ) ;
#12994=CARTESIAN_POINT ( 'NONE',  ( -10.85000000000000142, 2.500000000000000000, -5.802370205355746435 ) ) ;
#12995=DIRECTION ( 'NONE',  ( 0.000000000000000000, -0.9999939076577903929, 0.003490651415223739937 ) ) ;
#12996=FACE_BOUND ( 'NONE', #104435, .T. ) ;
#12997=DIRECTION ( 'NONE',  ( 0.000000000000000000, 0.000000000000000000, -1.000000000000000000 ) ) ;
#12998=FACE_OUTER_BOUND ( 'NONE', #12968, .T. ) ;
#12999=DIRECTION ( 'NONE',  ( -4.274815082592931898E-19, -0.9999939076577903929, -0.003490651415223739937 ) ) ;
#13001=PLANE ( 'NONE',  #52942 ) ;
#13002=DIRECTION ( 'NONE',  ( 0.000000000000000000, -0.9999939076577903929, 0.003490651415223739937 ) ) ;
#13003=ORIENTED_EDGE ( 'NONE', *, *, #90188, .F. ) ;
#13004=EDGE_CURVE ( 'NONE', #101973, #56674, #16522, .T. ) ;
#13005=CARTESIAN_POINT ( 'NONE',  ( 4.999999999999969802, 12.50000000000000000, 4.330127018922196314 ) ) ;
#13006=EDGE_LOOP ( 'NONE', ( #127270, #28784, #70697, #31091 ) ) ;
#13007=ORIENTED_EDGE ( 'NONE', *, *, #19931, .F. ) ;
#13008=DIRECTION ( 'NONE',  ( 0.000000000000000000, 0.000000000000000000, 1.000000000000000000 ) ) ;
#13009=EDGE_CURVE ( 'NONE', #38596, #49056, #43451, .T. ) ;
#13010=DIRECTION ( 'NONE',  ( 0.000000000000000000, -0.9999939076577903929, 0.003490651415223739937 ) ) ;
#13011=FACE_BOUND ( 'NONE', #119466, .T. ) ;
#13012=ADVANCED_FACE ( 'NONE', ( #64983 ), #60218, .T. ) ;
#13013=CARTESIAN_POINT ( 'NONE',  ( -1.900000000000035438, 12.50000000000000000, 3.983716857408420076 ) ) ;
#13014=AXIS2_PLACEMENT_3D ( 'NONE', #78157, #99083, #36306 ) ;
#13015=AXIS2_PLACEMENT_3D ( 'NONE', #103631, #53247, #51961 ) ;
#13016=EDGE_CURVE ( 'NONE', #34741, #58724, #120836, .T. ) ;
#13017=EDGE_CURVE ( 'NONE', #117086, #65795, #85235, .T. ) ;
#13018=EDGE_LOOP ( 'NONE', ( #3223, #23106 ) ) ;
#13019=CARTESIAN_POINT ( 'NONE',  ( 65.34954526967068489, 3.515384427023733327, 5.621991122696823773 ) ) ;
#13020=EDGE_CURVE ( 'NONE', #73744, #84243, #37221, .T. ) ;
#13021=EDGE_CURVE ( 'NONE', #94856, #70361, #97833, .T. ) ;
#13022=LINE ( 'NONE', #83092, #72847 ) ;
#13023=EDGE_CURVE ( 'NONE', #87315, #78724, #36201, .T. ) ;
#13024=ORIENTED_EDGE ( 'NONE', *, *, #35686, .T. ) ;
#13025=VECTOR ( 'NONE', #44571, 1000.000000000000000 ) ;
#13026=FACE_OUTER_BOUND ( 'NONE', #129219, .T. ) ;
#13027=PLANE ( 'NONE',  #63786 ) ;
#13028=AXIS2_PLACEMENT_3D ( 'NONE', #70823, #101582, #39466 ) ;
#13029=CIRCLE ( 'NONE', #86194, 0.06509327318403745899 ) ;
#13030=CIRCLE ( 'NONE', #86196, 0.1000000000000002554 ) ;
#13031=ORIENTED_EDGE ( 'NONE', *, *, #77174, .F. ) ;
#13032=DIRECTION ( 'NONE',  ( 0.000000000000000000, 0.000000000000000000, -1.000000000000000000 ) ) ;
#13033=DIRECTION ( 'NONE',  ( -0.000000000000000000, 1.000000000000000000, -0.000000000000000000 ) ) ;
#13034=EDGE_CURVE ( 'NONE', #35370, #32515, #116029, .T. ) ;
#13035=CONICAL_SURFACE ( 'NONE', #77996, 0.09999999999999999167, 0.003490658503988666988 ) ;
#13036=ORIENTED_EDGE ( 'NONE', *, *, #72533, .F. ) ;
#13037=DIRECTION ( 'NONE',  ( 0.000000000000000000, 1.000000000000000000, 0.000000000000000000 ) ) ;
#13038=CONICAL_SURFACE ( 'NONE', #117489, 0.1000000000000002554, 0.003490658503988666988 ) ;
#13039=DIRECTION ( 'NONE',  ( -0.000000000000000000, 1.000000000000000000, -0.000000000000000000 ) ) ;
#13040=DIRECTION ( 'NONE',  ( 0.000000000000000000, -0.9999939076577903929, 0.003490651415223739937 ) ) ;
#13041=ORIENTED_EDGE ( 'NONE', *, *, #18761, .F. ) ;
#13042=ORIENTED_EDGE ( 'NONE', *, *, #76448, .F. ) ;
#13044=EDGE_LOOP ( 'NONE', ( #46334, #7376 ) ) ;
#13045=CARTESIAN_POINT ( 'NONE',  ( -8.950000000000008171, 2.500000000000000000, 1.918653347947321564 ) ) ;
#13046=DIRECTION ( 'NONE',  ( 0.000000000000000000, -0.9999939076577903929, 0.003490651415223739937 ) ) ;
#13047=VERTEX_POINT ( 'NONE', #106220 ) ;
#13049=CARTESIAN_POINT ( 'NONE',  ( 11.84999999999990727, 2.500000000000000000, -2.411473670974877859 ) ) ;
#13050=CARTESIAN_POINT ( 'NONE',  ( 12.29999999999990123, 12.50000000000000000, 0.3464101615137735735 ) ) ;
#13051=CARTESIAN_POINT ( 'NONE',  ( -3.750000000000025757, 2.500000000000000000, -2.857883832488653741 ) ) ;
#13052=CIRCLE ( 'NONE', #102959, 0.09999999999999982514 ) ;
#13053=LINE ( 'NONE', #94864, #99690 ) ;
#13054=ORIENTED_EDGE ( 'NONE', *, *, #106885, .T. ) ;
#13055=ORIENTED_EDGE ( 'NONE', *, *, #22342, .F. ) ;
#13056=DIRECTION ( 'NONE',  ( 0.000000000000000000, 0.000000000000000000, 1.000000000000000000 ) ) ;
#13057=EDGE_LOOP ( 'NONE', ( #96920, #93253, #54424, #44278 ) ) ;
#13058=CIRCLE ( 'NONE', #100896, 0.09999999999999999167 ) ;
#13059=DIRECTION ( 'NONE',  ( 0.000000000000000000, -0.9999939076577903929, 0.003490651415223739937 ) ) ;
#13060=CIRCLE ( 'NONE', #46522, 0.06509327318403745899 ) ;
#13061=AXIS2_PLACEMENT_3D ( 'NONE', #87644, #10228, #7145 ) ;
#13062=EDGE_CURVE ( 'NONE', #16232, #79210, #74866, .T. ) ;
#13063=EDGE_LOOP ( 'NONE', ( #108632, #114549 ) ) ;
#13064=ORIENTED_EDGE ( 'NONE', *, *, #6304, .T. ) ;
#13065=VERTEX_POINT ( 'NONE', #4129 ) ;
#13066=EDGE_CURVE ( 'NONE', #62016, #96759, #78994, .T. ) ;
#13067=DIRECTION ( 'NONE',  ( -0.000000000000000000, 1.000000000000000000, -0.000000000000000000 ) ) ;
#13068=EDGE_CURVE ( 'NONE', #42458, #118390, #49748, .T. ) ;
#13069=DIRECTION ( 'NONE',  ( 0.000000000000000000, 1.000000000000000000, 0.000000000000000000 ) ) ;
#13070=CONICAL_SURFACE ( 'NONE', #11021, 0.1000000000000002554, 0.003490658503988666988 ) ;
#13071=CIRCLE ( 'NONE', #115473, 0.06509327318403745899 ) ;
#13072=FACE_OUTER_BOUND ( 'NONE', #50654, .T. ) ;
#13073=ADVANCED_FACE ( 'NONE', ( #56458 ), #7352, .T. ) ;
#13075=FACE_OUTER_BOUND ( 'NONE', #87613, .T. ) ;
#13076=CARTESIAN_POINT ( 'NONE',  ( -5.600000000000020073, 2.500000000000000000, 4.576537180435972019 ) ) ;
#13077=CARTESIAN_POINT ( 'NONE',  ( -0.6500000000000389910, 2.500000000000000000, -6.048780366869526581 ) ) ;
#13078=VECTOR ( 'NONE', #70882, 1000.000000000000000 ) ;
#13079=CARTESIAN_POINT ( 'NONE',  ( 3.349999999999945466, 12.50000000000000000, -2.165063509461101710 ) ) ;
#13080=CARTESIAN_POINT ( 'NONE',  ( -8.350000000000012079, 2.500000000000000000, -1.472243186433550122 ) ) ;
#13082=CARTESIAN_POINT ( 'NONE',  ( 7.899999999999924860, 2.500000000000000000, 4.922947341949748257 ) ) ;
#13083=CIRCLE ( 'NONE', #119705, 0.1000000000000002554 ) ;
#13084=EDGE_CURVE ( 'NONE', #39004, #121634, #26742, .T. ) ;
#13085=ADVANCED_FACE ( 'NONE', ( #97679 ), #87207, .T. ) ;
#13086=VERTEX_POINT ( 'NONE', #128456 ) ;
#13087=EDGE_CURVE ( 'NONE', #67710, #60176, #106841, .T. ) ;
#13088=CARTESIAN_POINT ( 'NONE',  ( -3.150000000000030553, 2.500000000000000000, 6.248780366869520542 ) ) ;
#13089=ORIENTED_EDGE ( 'NONE', *, *, #87692, .T. ) ;
#13090=EDGE_LOOP ( 'NONE', ( #110355, #46045, #48715, #127508 ) ) ;
#13091=LINE ( 'NONE', #93606, #33651 ) ;
#13092=CARTESIAN_POINT ( 'NONE',  ( -2.100000000000033396, 2.500000000000000000, -5.122947341949753763 ) ) ;
#13093=DIRECTION ( 'NONE',  ( 0.000000000000000000, -0.000000000000000000, 1.000000000000000000 ) ) ;
#13094=ADVANCED_FACE ( 'NONE', ( #76760 ), #10022, .T. ) ;
#13095=CIRCLE ( 'NONE', #50774, 0.09999999999999982514 ) ;
#13096=CARTESIAN_POINT ( 'NONE',  ( 12.89999999999989910, 12.50000000000000000, 0.6928203230275494784 ) ) ;
#13097=DIRECTION ( 'NONE',  ( -0.000000000000000000, 1.000000000000000000, -0.000000000000000000 ) ) ;
#13098=CARTESIAN_POINT ( 'NONE',  ( -5.400000000000019895, 2.500000000000000000, -2.276824562219559311E-15 ) ) ;
#13099=FACE_OUTER_BOUND ( 'NONE', #44753, .T. ) ;
#13100=EDGE_LOOP ( 'NONE', ( #68005, #22445 ) ) ;
#13101=VECTOR ( 'NONE', #36196, 1000.000000000000000 ) ;
#13102=AXIS2_PLACEMENT_3D ( 'NONE', #127352, #9504, #37681 ) ;
#13103=ORIENTED_EDGE ( 'NONE', *, *, #4044, .F. ) ;
#13104=AXIS2_PLACEMENT_3D ( 'NONE', #125723, #6576, #56988 ) ;
#13105=EDGE_LOOP ( 'NONE', ( #77767, #26936, #92010, #66197 ) ) ;
#13106=EDGE_LOOP ( 'NONE', ( #85851, #62775 ) ) ;
#13107=EDGE_CURVE ( 'NONE', #22575, #84951, #8003, .T. ) ;
#13108=EDGE_LOOP ( 'NONE', ( #117519, #9755 ) ) ;
#13109=VECTOR ( 'NONE', #99491, 1000.000000000000000 ) ;
#13110=CARTESIAN_POINT ( 'NONE',  ( 9.999999999999948486, 2.500000000000000000, -4.330127018922201643 ) ) ;
#13111=FACE_OUTER_BOUND ( 'NONE', #106105, .T. ) ;
#13113=CIRCLE ( 'NONE', #54987, 0.06509327318403745899 ) ;
#13114=CARTESIAN_POINT ( 'NONE',  ( 6.249999999999932498, 12.50000000000000000, -5.802370205355749988 ) ) ;
#13115=CONICAL_SURFACE ( 'NONE', #69564, 0.09999999999999999167, 0.003490658503988666988 ) ;
#13116=DIRECTION ( 'NONE',  ( 0.000000000000000000, 0.000000000000000000, 1.000000000000000000 ) ) ;
#13117=DIRECTION ( 'NONE',  ( 0.000000000000000000, 1.000000000000000000, 0.000000000000000000 ) ) ;
#13119=CARTESIAN_POINT ( 'NONE',  ( 43.31340628060505793, -2.029328412884075838, 5.113049426574150402 ) ) ;
#13120=DIRECTION ( 'NONE',  ( 0.000000000000000000, 0.000000000000000000, 1.000000000000000000 ) ) ;
#13121=CARTESIAN_POINT ( 'NONE',  ( -3.300000000000027800, 12.50000000000000000, 0.06509327318403515528 ) ) ;
#13122=AXIS2_PLACEMENT_3D ( 'NONE', #52958, #41856, #81752 ) ;
#13123=AXIS2_PLACEMENT_3D ( 'NONE', #56329, #116546, #115226 ) ;
#13124=DIRECTION ( 'NONE',  ( -0.000000000000000000, -1.000000000000000000, -0.000000000000000000 ) ) ;
#13125=VERTEX_POINT ( 'NONE', #28302 ) ;
#13126=EDGE_CURVE ( 'NONE', #20627, #69676, #22650, .T. ) ;
#13127=CONICAL_SURFACE ( 'NONE', #98819, 0.1000000000000002554, 0.003490658503988666988 ) ;
#13129=ORIENTED_EDGE ( 'NONE', *, *, #113398, .F. ) ;
#13130=EDGE_LOOP ( 'NONE', ( #25654, #99192, #122534, #87896 ) ) ;
#13131=DIRECTION ( 'NONE',  ( 0.000000000000000000, -0.9999939076577903929, 0.003490651415223739937 ) ) ;
#13132=CIRCLE ( 'NONE', #94716, 0.06509327318403745899 ) ;
#13133=CARTESIAN_POINT ( 'NONE',  ( 4.999999999999936939, 2.500000000000000000, -0.7928203230275542301 ) ) ;
#13134=LINE ( 'NONE', #14424, #10524 ) ;
#13135=CIRCLE ( 'NONE', #29885, 0.1000000000000000472 ) ;
#13136=VERTEX_POINT ( 'NONE', #9301 ) ;
#13137=DIRECTION ( 'NONE',  ( 0.000000000000000000, 1.000000000000000000, 0.000000000000000000 ) ) ;
#13138=CARTESIAN_POINT ( 'NONE',  ( -3.350000000000028955, 12.50000000000000000, 2.230156782645134950 ) ) ;
#13140=DIRECTION ( 'NONE',  ( 0.000000000000000000, -0.000000000000000000, 1.000000000000000000 ) ) ;
#13141=PLANE ( 'NONE',  #66492 ) ;
#13142=DIRECTION ( 'NONE',  ( -0.000000000000000000, -1.000000000000000000, -0.000000000000000000 ) ) ;
#13143=VERTEX_POINT ( 'NONE', #27630 ) ;
#13144=AXIS2_PLACEMENT_3D ( 'NONE', #24858, #23566, #64772 ) ;
#13145=EDGE_LOOP ( 'NONE', ( #88927, #44891 ) ) ;
#13146=CIRCLE ( 'NONE', #73801, 0.1000000000000002554 ) ;
#13147=CARTESIAN_POINT ( 'NONE',  ( -1.900000000000035438, 2.500000000000000000, 4.083716857408420609 ) ) ;
#13148=DIRECTION ( 'NONE',  ( -0.000000000000000000, 1.000000000000000000, -0.000000000000000000 ) ) ;
#13149=DIRECTION ( 'NONE',  ( -0.000000000000000000, -1.000000000000000000, -0.000000000000000000 ) ) ;
#13150=DIRECTION ( 'NONE',  ( -0.000000000000000000, 1.000000000000000000, -0.000000000000000000 ) ) ;
#13151=EDGE_LOOP ( 'NONE', ( #95718, #99214, #121649, #32479 ) ) ;
#13152=AXIS2_PLACEMENT_3D ( 'NONE', #90754, #32511, #119560 ) ;
#13153=CIRCLE ( 'NONE', #29912, 0.1000000000000002554 ) ;
#13154=CIRCLE ( 'NONE', #42446, 0.1000000000000000472 ) ;
#13155=ORIENTED_EDGE ( 'NONE', *, *, #78972, .T. ) ;
#13156=PLANE ( 'NONE',  #125371 ) ;
#13157=DIRECTION ( 'NONE',  ( 0.000000000000000000, -0.9999939076577903929, 0.003490651415223739937 ) ) ;
#13158=PLANE ( 'NONE',  #82083 ) ;
#13159=CARTESIAN_POINT ( 'NONE',  ( -6.450000000000019718, 2.500000000000000000, -6.148780366869526226 ) ) ;
#13160=CARTESIAN_POINT ( 'NONE',  ( 4.999999999999973355, 2.500000000000000000, -4.230127018922201998 ) ) ;
#13161=VERTEX_POINT ( 'NONE', #86565 ) ;
#13162=CIRCLE ( 'NONE', #59173, 0.06509327318403745899 ) ;
#13163=DIRECTION ( 'NONE',  ( -0.000000000000000000, 1.000000000000000000, -0.000000000000000000 ) ) ;
#13164=ADVANCED_FACE ( 'NONE', ( #8633 ), #60311, .T. ) ;
#13165=CARTESIAN_POINT ( 'NONE',  ( -10.40000000000000213, 2.500000000000000000, 0.6928203230275494784 ) ) ;
#13166=AXIS2_PLACEMENT_3D ( 'NONE', #120310, #110481, #20819 ) ;
#13167=EDGE_LOOP ( 'NONE', ( #102118, #26859, #85353, #100914 ) ) ;
#13168=DIRECTION ( 'NONE',  ( 0.000000000000000000, 0.000000000000000000, -1.000000000000000000 ) ) ;
#13169=ORIENTED_EDGE ( 'NONE', *, *, #38468, .T. ) ;
#13170=VECTOR ( 'NONE', #78008, 1000.000000000000000 ) ;
#13171=CARTESIAN_POINT ( 'NONE',  ( -1.700000000000034817, 12.50000000000000000, -4.330127018922201643 ) ) ;
#13172=VERTEX_POINT ( 'NONE', #78705 ) ;
#13173=DIRECTION ( 'NONE',  ( 0.000000000000000000, 1.000000000000000000, 0.000000000000000000 ) ) ;
#13174=CARTESIAN_POINT ( 'NONE',  ( 6.649999999999928413, 2.500000000000000000, 1.572243186433545548 ) ) ;
#13175=ADVANCED_FACE ( 'NONE', ( #127784 ), #119248, .T. ) ;
#13176=EDGE_LOOP ( 'NONE', ( #79654, #67909, #16343, #73857 ) ) ;
#13177=ADVANCED_FACE ( 'NONE', ( #38792 ), #39389, .T. ) ;
#13178=VERTEX_POINT ( 'NONE', #19092 ) ;
#13179=EDGE_CURVE ( 'NONE', #49764, #179, #59054, .T. ) ;
#13180=EDGE_CURVE ( 'NONE', #49224, #43749, #129107, .T. ) ;
#13183=AXIS2_PLACEMENT_3D ( 'NONE', #56467, #77412, #67571 ) ;
#13184=DIRECTION ( 'NONE',  ( 0.000000000000000000, 0.000000000000000000, -1.000000000000000000 ) ) ;
#13185=CARTESIAN_POINT ( 'NONE',  ( 5.399999999999936406, 12.50000000000000000, -5.022947341949754119 ) ) ;
#13187=DIRECTION ( 'NONE',  ( 0.000000000000000000, 1.000000000000000000, 0.000000000000000000 ) ) ;
#13188=CARTESIAN_POINT ( 'NONE',  ( -5.600000000000020073, 12.50000000000000000, -0.3464101615137782364 ) ) ;
#13189=CARTESIAN_POINT ( 'NONE',  ( 9.199999999999915801, 12.50000000000000000, -4.395220292106239768 ) ) ;
#13190=CARTESIAN_POINT ( 'NONE',  ( -5.400000000000020783, 12.50000000000000000, 4.957854068765711553 ) ) ;
#13191=EDGE_CURVE ( 'NONE', #3245, #40491, #110451, .T. ) ;
#13192=VECTOR ( 'NONE', #90918, 1000.000000000000000 ) ;
#13193=AXIS2_PLACEMENT_3D ( 'NONE', #106256, #116069, #33654 ) ;
#13194=EDGE_CURVE ( 'NONE', #104331, #121408, #45632, .T. ) ;
#13195=CIRCLE ( 'NONE', #92638, 0.1000000000000002554 ) ;
#13196=ADVANCED_FACE ( 'NONE', ( #30256 ), #49839, .T. ) ;
#13197=VERTEX_POINT ( 'NONE', #79970 ) ;
#13198=VERTEX_POINT ( 'NONE', #120545 ) ;
#13199=DIRECTION ( 'NONE',  ( 0.000000000000000000, 1.000000000000000000, 0.000000000000000000 ) ) ;
#13200=EDGE_LOOP ( 'NONE', ( #14637, #98227, #73551, #51717 ) ) ;
#13201=LINE ( 'NONE', #102871, #28693 ) ;
#13202=CARTESIAN_POINT ( 'NONE',  ( -1.650000000000034328, 12.50000000000000000, -7.188010851410854052 ) ) ;
#13203=DIRECTION ( 'NONE',  ( 0.000000000000000000, 0.000000000000000000, 1.000000000000000000 ) ) ;
#13204=ORIENTED_EDGE ( 'NONE', *, *, #97767, .T. ) ;
#13205=ORIENTED_EDGE ( 'NONE', *, *, #108921, .F. ) ;
#13206=FACE_BOUND ( 'NONE', #116516, .T. ) ;
#13207=EDGE_LOOP ( 'NONE', ( #11206, #61153 ) ) ;
#13208=CIRCLE ( 'NONE', #90581, 0.1000000000000002554 ) ;
#13209=CARTESIAN_POINT ( 'NONE',  ( -0.4500000000000402012, 12.50000000000000000, 2.165063509461097713 ) ) ;
#13210=CARTESIAN_POINT ( 'NONE',  ( -1.900000000000034994, 2.500000000000000000, -4.576537180435978236 ) ) ;
#13211=AXIS2_PLACEMENT_3D ( 'NONE', #127425, #128739, #77028 ) ;
#13212=FACE_OUTER_BOUND ( 'NONE', #69238, .T. ) ;
#13213=PLANE ( 'NONE',  #7512 ) ;
#13214=AXIS2_PLACEMENT_3D ( 'NONE', #104734, #109082, #115186 ) ;
#13215=DIRECTION ( 'NONE',  ( 0.000000000000000000, 0.000000000000000000, 1.000000000000000000 ) ) ;
#13216=FACE_OUTER_BOUND ( 'NONE', #36004, .T. ) ;
#13217=DIRECTION ( 'NONE',  ( 0.000000000000000000, 0.000000000000000000, 1.000000000000000000 ) ) ;
#13218=DIRECTION ( 'NONE',  ( -4.274815082592931898E-19, -0.9999939076577903929, -0.003490651415223739937 ) ) ;
#13219=DIRECTION ( 'NONE',  ( 0.000000000000000000, -0.9999939076577903929, 0.003490651415223739937 ) ) ;
#13220=DIRECTION ( 'NONE',  ( 0.000000000000000000, 0.000000000000000000, 1.000000000000000000 ) ) ;
#13221=DIRECTION ( 'NONE',  ( -0.000000000000000000, -1.000000000000000000, -0.000000000000000000 ) ) ;
#13222=ORIENTED_EDGE ( 'NONE', *, *, #121521, .F. ) ;
#13223=ORIENTED_EDGE ( 'NONE', *, *, #30499, .T. ) ;
#13224=ORIENTED_EDGE ( 'NONE', *, *, #21382, .T. ) ;
#13225=CARTESIAN_POINT ( 'NONE',  ( 10.39999999999990976, 2.500000000000000000, 4.430127018922196847 ) ) ;
#13226=ORIENTED_EDGE ( 'NONE', *, *, #28444, .F. ) ;
#13227=DIRECTION ( 'NONE',  ( 0.000000000000000000, 0.000000000000000000, 1.000000000000000000 ) ) ;
#13229=EDGE_LOOP ( 'NONE', ( #28765, #7941 ) ) ;
#13230=EDGE_LOOP ( 'NONE', ( #58246, #90153, #56548, #127801 ) ) ;
#13231=CIRCLE ( 'NONE', #119855, 0.06509327318403745899 ) ;
#13233=DIRECTION ( 'NONE',  ( -4.274815082592931898E-19, -0.9999939076577903929, -0.003490651415223739937 ) ) ;
#13234=FACE_OUTER_BOUND ( 'NONE', #76372, .T. ) ;
#13236=CARTESIAN_POINT ( 'NONE',  ( -9.400000000000007461, 2.500000000000000000, 0.4464101615137735513 ) ) ;
#13237=ORIENTED_EDGE ( 'NONE', *, *, #46171, .F. ) ;
#13238=EDGE_CURVE ( 'NONE', #10798, #123447, #58247, .T. ) ;
#13239=DIRECTION ( 'NONE',  ( 0.000000000000000000, 0.000000000000000000, 1.000000000000000000 ) ) ;
#13240=ORIENTED_EDGE ( 'NONE', *, *, #94451, .T. ) ;
#13241=ADVANCED_FACE ( 'NONE', ( #99624 ), #122988, .T. ) ;
#13242=ORIENTED_EDGE ( 'NONE', *, *, #82237, .F. ) ;
#13243=ORIENTED_EDGE ( 'NONE', *, *, #108724, .T. ) ;
#13244=ADVANCED_FACE ( 'NONE', ( #112 ), #20417, .T. ) ;
#13245=FACE_OUTER_BOUND ( 'NONE', #17994, .T. ) ;
#13246=CIRCLE ( 'NONE', #80161, 0.09999999999999982514 ) ;
#13247=AXIS2_PLACEMENT_3D ( 'NONE', #118205, #88747, #67139 ) ;
#13248=VERTEX_POINT ( 'NONE', #22362 ) ;
#13250=ORIENTED_EDGE ( 'NONE', *, *, #82726, .T. ) ;
#13252=ADVANCED_FACE ( 'NONE', ( #41362 ), #81223, .T. ) ;
#13253=CIRCLE ( 'NONE', #86414, 0.06509327318403741736 ) ;
#13254=DIRECTION ( 'NONE',  ( 0.000000000000000000, 0.000000000000000000, 1.000000000000000000 ) ) ;
#13255=AXIS2_PLACEMENT_3D ( 'NONE', #721, #58380, #77999 ) ;
#13256=FACE_OUTER_BOUND ( 'NONE', #54597, .T. ) ;
#13257=CONICAL_SURFACE ( 'NONE', #71867, 0.1000000000000000056, 0.003490658503988666988 ) ;
#13258=LINE ( 'NONE', #74780, #96505 ) ;
#13260=AXIS2_PLACEMENT_3D ( 'NONE', #102581, #71856, #12898 ) ;
#13261=CIRCLE ( 'NONE', #50944, 0.09999999999999982514 ) ;
#13262=DIRECTION ( 'NONE',  ( -4.274815082592931898E-19, -0.9999939076577903929, -0.003490651415223739937 ) ) ;
#13263=FACE_OUTER_BOUND ( 'NONE', #104039, .T. ) ;
#13264=AXIS2_PLACEMENT_3D ( 'NONE', #30083, #107976, #88983 ) ;
#13265=AXIS2_PLACEMENT_3D ( 'NONE', #41448, #82653, #81366 ) ;
#13267=CARTESIAN_POINT ( 'NONE',  ( -10.00000000000000711, 12.50000000000000000, -3.637306695894645614 ) ) ;
#13268=CIRCLE ( 'NONE', #103162, 0.09999999999999999167 ) ;
#13269=ORIENTED_EDGE ( 'NONE', *, *, #66892, .F. ) ;
#13271=VECTOR ( 'NONE', #14828, 1000.000000000000000 ) ;
#13272=ORIENTED_EDGE ( 'NONE', *, *, #6706, .T. ) ;
#13273=VECTOR ( 'NONE', #26969, 1000.000000000000000 ) ;
#13274=VERTEX_POINT ( 'NONE', #50505 ) ;
#13275=CARTESIAN_POINT ( 'NONE',  ( -11.84999999999999787, 12.50000000000000000, -6.148780366869522673 ) ) ;
#13277=CARTESIAN_POINT ( 'NONE',  ( 5.599999999999933031, 2.500000000000000000, -0.4464101615137783252 ) ) ;
#13278=ORIENTED_EDGE ( 'NONE', *, *, #65843, .F. ) ;
#13279=ORIENTED_EDGE ( 'NONE', *, *, #53103, .T. ) ;
#13280=FACE_OUTER_BOUND ( 'NONE', #88634, .T. ) ;
#13281=DIRECTION ( 'NONE',  ( -0.000000000000000000, -1.000000000000000000, -0.000000000000000000 ) ) ;
#13282=CARTESIAN_POINT ( 'NONE',  ( -8.950000000000009948, 2.500000000000000000, -1.818653347947326138 ) ) ;
#13283=DIRECTION ( 'NONE',  ( 0.000000000000000000, 0.000000000000000000, -1.000000000000000000 ) ) ;
#13284=AXIS2_PLACEMENT_3D ( 'NONE', #109448, #110093, #89804 ) ;
#13285=DIRECTION ( 'NONE',  ( 0.000000000000000000, 0.000000000000000000, 1.000000000000000000 ) ) ;
#13286=EDGE_LOOP ( 'NONE', ( #5465, #122974 ) ) ;
#13287=EDGE_CURVE ( 'NONE', #39657, #82277, #24786, .T. ) ;
#13288=DIRECTION ( 'NONE',  ( 0.000000000000000000, 0.000000000000000000, -1.000000000000000000 ) ) ;
#13289=CIRCLE ( 'NONE', #4971, 0.1000000000000002554 ) ;
#13290=VERTEX_POINT ( 'NONE', #32825 ) ;
#13291=CIRCLE ( 'NONE', #34258, 0.06509327318403745899 ) ;
#13292=PLANE ( 'NONE',  #59119 ) ;
#13293=DIRECTION ( 'NONE',  ( 0.000000000000000000, 0.000000000000000000, 1.000000000000000000 ) ) ;
#13294=AXIS2_PLACEMENT_3D ( 'NONE', #116839, #37664, #46840 ) ;
#13295=EDGE_CURVE ( 'NONE', #33480, #43682, #62282, .T. ) ;
#13297=CARTESIAN_POINT ( 'NONE',  ( 6.249999999999965361, 12.50000000000000000, 2.230156782645134950 ) ) ;
#13298=CARTESIAN_POINT ( 'NONE',  ( 0.3999999999999568345, 2.500000000000000000, -3.637306695894650055 ) ) ;
#13299=ADVANCED_FACE ( 'NONE', ( #70797 ), #129268, .T. ) ;
#13300=DIRECTION ( 'NONE',  ( -4.274815082592931898E-19, -0.9999939076577903929, -0.003490651415223739937 ) ) ;
#13301=CIRCLE ( 'NONE', #109458, 0.1000000000000002554 ) ;
#13302=CARTESIAN_POINT ( 'NONE',  ( 6.249999999999930722, 2.500000000000000000, -1.372243186433550033 ) ) ;
#13303=AXIS2_PLACEMENT_3D ( 'NONE', #60631, #23250, #110977 ) ;
#13304=ORIENTED_EDGE ( 'NONE', *, *, #128052, .F. ) ;
#13305=AXIS2_PLACEMENT_3D ( 'NONE', #81513, #121419, #1009 ) ;
#13306=CONICAL_SURFACE ( 'NONE', #67690, 0.09999999999999982514, 0.003490658503988666988 ) ;
#13307=DIRECTION ( 'NONE',  ( -0.000000000000000000, -1.000000000000000000, -0.000000000000000000 ) ) ;
#13308=DIRECTION ( 'NONE',  ( 0.000000000000000000, 0.000000000000000000, 1.000000000000000000 ) ) ;
#13309=CARTESIAN_POINT ( 'NONE',  ( 3.299999999999942979, 12.50000000000000000, 4.330127018922196314 ) ) ;
#13310=VERTEX_POINT ( 'NONE', #82568 ) ;
#13311=ADVANCED_FACE ( 'NONE', ( #81270 ), #120919, .T. ) ;
#13312=AXIS2_PLACEMENT_3D ( 'NONE', #99858, #67802, #99212 ) ;
#13313=CARTESIAN_POINT ( 'NONE',  ( -6.850000000000013856, 12.50000000000000000, 1.883746621131358934 ) ) ;
#13314=ORIENTED_EDGE ( 'NONE', *, *, #123574, .T. ) ;
#13315=AXIS2_PLACEMENT_3D ( 'NONE', #83380, #123294, #80806 ) ;
#13316=AXIS2_PLACEMENT_3D ( 'NONE', #38006, #38678, #19661 ) ;
#13317=VERTEX_POINT ( 'NONE', #122486 ) ;
#13318=CIRCLE ( 'NONE', #55108, 0.1000000000000002554 ) ;
#13319=PLANE ( 'NONE',  #94836 ) ;
#13320=ORIENTED_EDGE ( 'NONE', *, *, #3449, .T. ) ;
#13321=CARTESIAN_POINT ( 'NONE',  ( 17.33812564108167109, -2.538896947916728042, -5.379288978446362890 ) ) ;
#13322=DIRECTION ( 'NONE',  ( -0.000000000000000000, 1.000000000000000000, -0.000000000000000000 ) ) ;
#13323=CARTESIAN_POINT ( 'NONE',  ( 2.099999999999949463, 2.500000000000000000, -3.637306695894650055 ) ) ;
#13324=CIRCLE ( 'NONE', #103230, 0.06509327318403745899 ) ;
#13325=ORIENTED_EDGE ( 'NONE', *, *, #60721, .T. ) ;
#13326=FACE_OUTER_BOUND ( 'NONE', #14209, .T. ) ;
#13327=EDGE_CURVE ( 'NONE', #99644, #83794, #9946, .T. ) ;
#13328=CARTESIAN_POINT ( 'NONE',  ( 9.399999999999915090, 2.500000000000000000, -4.676537180435977881 ) ) ;
#13329=EDGE_LOOP ( 'NONE', ( #51943, #22724, #7559, #798 ) ) ;
#13330=EDGE_CURVE ( 'NONE', #95574, #120916, #37315, .T. ) ;
#13331=EDGE_LOOP ( 'NONE', ( #35059, #83982, #36088, #48029 ) ) ;
#13332=EDGE_LOOP ( 'NONE', ( #98087, #4659 ) ) ;
#13333=DIRECTION ( 'NONE',  ( -0.000000000000000000, -1.000000000000000000, -0.000000000000000000 ) ) ;
#13334=DIRECTION ( 'NONE',  ( 0.000000000000000000, 1.000000000000000000, 0.000000000000000000 ) ) ;
#13335=AXIS2_PLACEMENT_3D ( 'NONE', #114364, #86171, #97312 ) ;
#13336=CARTESIAN_POINT ( 'NONE',  ( -5.800000000000018474, 12.50000000000000000, -2.276824562219559311E-15 ) ) ;
#13337=EDGE_CURVE ( 'NONE', #124980, #75076, #93740, .T. ) ;
#13338=AXIS2_PLACEMENT_3D ( 'NONE', #55569, #113850, #83739 ) ;
#13339=ADVANCED_FACE ( 'NONE', ( #761 ), #106254, .T. ) ;
#13340=ORIENTED_EDGE ( 'NONE', *, *, #112615, .T. ) ;
#13341=EDGE_CURVE ( 'NONE', #55354, #18200, #66534, .T. ) ;
#13342=EDGE_CURVE ( 'NONE', #46558, #36089, #43930, .T. ) ;
#13343=DIRECTION ( 'NONE',  ( 0.000000000000000000, 0.000000000000000000, -1.000000000000000000 ) ) ;
#13344=DIRECTION ( 'NONE',  ( 0.000000000000000000, 0.000000000000000000, 1.000000000000000000 ) ) ;
#13345=ORIENTED_EDGE ( 'NONE', *, *, #31233, .F. ) ;
#13346=DIRECTION ( 'NONE',  ( 0.000000000000000000, -0.9999939076577903929, 0.003490651415223739937 ) ) ;
#13347=DIRECTION ( 'NONE',  ( 0.000000000000000000, 0.000000000000000000, 1.000000000000000000 ) ) ;
#13348=CIRCLE ( 'NONE', #117903, 0.1000000000000000472 ) ;
#13349=AXIS2_PLACEMENT_3D ( 'NONE', #97185, #7504, #47446 ) ;
#13350=VECTOR ( 'NONE', #89402, 1000.000000000000000 ) ;
#13351=EDGE_CURVE ( 'NONE', #17483, #90021, #94961, .T. ) ;
#13352=FACE_OUTER_BOUND ( 'NONE', #71155, .T. ) ;
#13353=CARTESIAN_POINT ( 'NONE',  ( 2.500000000000002220, -0.5000000000000004441, 10.00000000000000178 ) ) ;
#13354=CARTESIAN_POINT ( 'NONE',  ( -15.59999999999998010, 12.50000000000000000, -0.3464101615137759604 ) ) ;
#13355=ADVANCED_FACE ( 'NONE', ( #94291 ), #28905, .T. ) ;
#13356=CARTESIAN_POINT ( 'NONE',  ( 7.099999999999926814, 12.50000000000000000, 0.06509327318403515528 ) ) ;
#13357=CARTESIAN_POINT ( 'NONE',  ( -5.400000000000019895, 12.50000000000000000, 4.330127018922196314 ) ) ;
#13358=AXIS2_PLACEMENT_3D ( 'NONE', #14273, #83676, #113124 ) ;
#13359=EDGE_CURVE ( 'NONE', #79439, #109003, #83283, .T. ) ;
#13360=CIRCLE ( 'NONE', #113732, 0.06509327318403745899 ) ;
#13361=CIRCLE ( 'NONE', #78230, 0.09999999999999982514 ) ;
#13362=EDGE_CURVE ( 'NONE', #92091, #112676, #108397, .T. ) ;
#13363=EDGE_LOOP ( 'NONE', ( #85085, #88230, #96699, #60951 ) ) ;
#13364=ORIENTED_EDGE ( 'NONE', *, *, #21014, .T. ) ;
#13366=VERTEX_POINT ( 'NONE', #73367 ) ;
#13367=DIRECTION ( 'NONE',  ( 0.000000000000000000, -0.000000000000000000, 1.000000000000000000 ) ) ;
#13368=CARTESIAN_POINT ( 'NONE',  ( -9.400000000000009237, 2.500000000000000000, -3.883716857408422207 ) ) ;
#13369=DIRECTION ( 'NONE',  ( -0.000000000000000000, -1.000000000000000000, -0.000000000000000000 ) ) ;
#13370=EDGE_LOOP ( 'NONE', ( #20518, #3828 ) ) ;
#13371=EDGE_CURVE ( 'NONE', #5489, #27768, #26838, .T. ) ;
#13372=FACE_BOUND ( 'NONE', #62739, .T. ) ;
#13373=EDGE_CURVE ( 'NONE', #21305, #12208, #100002, .T. ) ;
#13374=DIRECTION ( 'NONE',  ( 0.000000000000000000, -0.000000000000000000, 1.000000000000000000 ) ) ;
#13375=FACE_OUTER_BOUND ( 'NONE', #59574, .T. ) ;
#13376=DIRECTION ( 'NONE',  ( 0.000000000000000000, 0.000000000000000000, -1.000000000000000000 ) ) ;
#13377=DIRECTION ( 'NONE',  ( 0.000000000000000000, 0.000000000000000000, 1.000000000000000000 ) ) ;
#13378=CARTESIAN_POINT ( 'NONE',  ( -3.350000000000029399, 2.500000000000000000, 6.595190528383296780 ) ) ;
#13379=DIRECTION ( 'NONE',  ( -0.000000000000000000, -1.000000000000000000, -0.000000000000000000 ) ) ;
#13380=DIRECTION ( 'NONE',  ( 0.000000000000000000, 0.000000000000000000, -1.000000000000000000 ) ) ;
#13381=CARTESIAN_POINT ( 'NONE',  ( 5.449999999999936229, 2.500000000000000000, 6.595190528383296780 ) ) ;
#13382=CARTESIAN_POINT ( 'NONE',  ( 13.54999999999990123, 12.50000000000000000, 1.818653347947321475 ) ) ;
#13383=VECTOR ( 'NONE', #6976, 1000.000000000000000 ) ;
#13384=ORIENTED_EDGE ( 'NONE', *, *, #22244, .F. ) ;
#13385=VERTEX_POINT ( 'NONE', #24925 ) ;
#13386=ORIENTED_EDGE ( 'NONE', *, *, #79697, .T. ) ;
#13387=ORIENTED_EDGE ( 'NONE', *, *, #26530, .T. ) ;
#13388=EDGE_LOOP ( 'NONE', ( #114877, #39822 ) ) ;
#13389=ORIENTED_EDGE ( 'NONE', *, *, #66031, .F. ) ;
#13390=DIRECTION ( 'NONE',  ( 0.000000000000000000, -0.000000000000000000, 1.000000000000000000 ) ) ;
#13391=ORIENTED_EDGE ( 'NONE', *, *, #6410, .F. ) ;
#13392=EDGE_LOOP ( 'NONE', ( #91136, #86358, #66497, #36149 ) ) ;
#13393=AXIS2_PLACEMENT_3D ( 'NONE', #116556, #119617, #89521 ) ;
#13394=CARTESIAN_POINT ( 'NONE',  ( 13.12246079397647236, -2.500000000000000444, 7.156134182876034977 ) ) ;
#13395=DIRECTION ( 'NONE',  ( -0.000000000000000000, 1.000000000000000000, -0.000000000000000000 ) ) ;
#13396=DIRECTION ( 'NONE',  ( 0.000000000000000000, -0.000000000000000000, 1.000000000000000000 ) ) ;
#13397=CONICAL_SURFACE ( 'NONE', #590, 0.1000000000000002554, 0.003490658503988666988 ) ;
#13398=ORIENTED_EDGE ( 'NONE', *, *, #31029, .T. ) ;
#13399=DIRECTION ( 'NONE',  ( 0.000000000000000000, 0.000000000000000000, -1.000000000000000000 ) ) ;
#13400=VERTEX_POINT ( 'NONE', #62912 ) ;
#13401=CONICAL_SURFACE ( 'NONE', #86563, 0.1000000000000002554, 0.003490658503988666988 ) ;
#13402=ADVANCED_FACE ( 'NONE', ( #53734 ), #93663, .T. ) ;
#13403=EDGE_LOOP ( 'NONE', ( #90667, #38687, #114327, #22421 ) ) ;
#13404=DIRECTION ( 'NONE',  ( -0.000000000000000000, 1.000000000000000000, -0.000000000000000000 ) ) ;
#13405=EDGE_CURVE ( 'NONE', #4060, #114757, #43585, .T. ) ;
#13406=DIRECTION ( 'NONE',  ( 0.000000000000000000, 1.000000000000000000, 0.000000000000000000 ) ) ;
#13407=EDGE_LOOP ( 'NONE', ( #3466, #8451 ) ) ;
#13408=ORIENTED_EDGE ( 'NONE', *, *, #83127, .T. ) ;
#13409=LINE ( 'NONE', #115459, #35934 ) ;
#13410=DIRECTION ( 'NONE',  ( 0.000000000000000000, 0.000000000000000000, 1.000000000000000000 ) ) ;
#13411=CONICAL_SURFACE ( 'NONE', #15553, 0.09999999999999982514, 0.003490658503988666988 ) ;
#13412=CARTESIAN_POINT ( 'NONE',  ( 3.349999999999943689, 2.500000000000000000, 1.472243186433545459 ) ) ;
#13413=AXIS2_PLACEMENT_3D ( 'NONE', #31421, #102088, #52988 ) ;
#13414=AXIS2_PLACEMENT_3D ( 'NONE', #99877, #20026, #111620 ) ;
#13415=DIRECTION ( 'NONE',  ( 0.000000000000000000, 0.000000000000000000, 1.000000000000000000 ) ) ;
#13416=CARTESIAN_POINT ( 'NONE',  ( -6.249999999999984901, 2.500000000000000000, -2.065063509461102065 ) ) ;
#13417=AXIS2_PLACEMENT_3D ( 'NONE', #85962, #15932, #55870 ) ;
#13418=EDGE_LOOP ( 'NONE', ( #123746, #35138, #13748, #124316 ) ) ;
#13419=CIRCLE ( 'NONE', #2974, 0.09999999999999999167 ) ;
#13420=DIRECTION ( 'NONE',  ( -0.000000000000000000, 1.000000000000000000, -0.000000000000000000 ) ) ;
#13421=ORIENTED_EDGE ( 'NONE', *, *, #62308, .F. ) ;
#13424=CARTESIAN_POINT ( 'NONE',  ( 15.59999999999988951, 2.500000000000000000, 0.2464101615137735679 ) ) ;
#13425=CARTESIAN_POINT ( 'NONE',  ( -6.050000000000020250, 12.50000000000000000, -2.511473670974877948 ) ) ;
#13426=DIRECTION ( 'NONE',  ( -0.000000000000000000, 1.000000000000000000, -0.000000000000000000 ) ) ;
#13427=FACE_OUTER_BOUND ( 'NONE', #16601, .T. ) ;
#13428=VERTEX_POINT ( 'NONE', #114575 ) ;
#13429=FACE_OUTER_BOUND ( 'NONE', #31524, .T. ) ;
#13430=CIRCLE ( 'NONE', #30190, 0.06509327318403745899 ) ;
#13432=DIRECTION ( 'NONE',  ( -0.000000000000000000, 1.000000000000000000, -0.000000000000000000 ) ) ;
#13434=ORIENTED_EDGE ( 'NONE', *, *, #39714, .F. ) ;
#13435=CIRCLE ( 'NONE', #99136, 0.09999999999999982514 ) ;
#13436=CIRCLE ( 'NONE', #109603, 0.06509327318403745899 ) ;
#13437=EDGE_LOOP ( 'NONE', ( #74422, #23551 ) ) ;
#13438=LINE ( 'NONE', #43578, #58330 ) ;
#13439=DIRECTION ( 'NONE',  ( -4.274815082592931898E-19, -0.9999939076577903929, -0.003490651415223739937 ) ) ;
#13441=DIRECTION ( 'NONE',  ( 0.000000000000000000, 1.000000000000000000, 0.000000000000000000 ) ) ;
#13442=DIRECTION ( 'NONE',  ( -0.000000000000000000, 1.000000000000000000, -0.000000000000000000 ) ) ;
#13443=EDGE_CURVE ( 'NONE', #38221, #108534, #72900, .T. ) ;
#13444=AXIS2_PLACEMENT_3D ( 'NONE', #92881, #112516, #22217 ) ;
#13445=DIRECTION ( 'NONE',  ( 0.000000000000000000, 0.000000000000000000, 1.000000000000000000 ) ) ;
#13446=AXIS2_PLACEMENT_3D ( 'NONE', #55177, #95104, #83973 ) ;
#13447=DIRECTION ( 'NONE',  ( 0.000000000000000000, 0.000000000000000000, 1.000000000000000000 ) ) ;
#13448=VERTEX_POINT ( 'NONE', #74023 ) ;
#13449=AXIS2_PLACEMENT_3D ( 'NONE', #73211, #43769, #116339 ) ;
#13450=AXIS2_PLACEMENT_3D ( 'NONE', #9740, #117735, #79142 ) ;
#13451=CARTESIAN_POINT ( 'NONE',  ( -12.49999999999999289, 2.500000000000000000, -5.022947341949751454 ) ) ;
#13452=VECTOR ( 'NONE', #88367, 1000.000000000000000 ) ;
#13453=EDGE_LOOP ( 'NONE', ( #48996, #39643 ) ) ;
#13454=DIRECTION ( 'NONE',  ( 0.000000000000000000, 1.000000000000000000, 0.000000000000000000 ) ) ;
#13455=CIRCLE ( 'NONE', #59467, 0.1000000000000002554 ) ;
#13456=ADVANCED_FACE ( 'NONE', ( #24272 ), #16434, .T. ) ;
#13457=CARTESIAN_POINT ( 'NONE',  ( -5.800000000000018474, 12.50000000000000000, -2.276824562219559311E-15 ) ) ;
#13458=EDGE_CURVE ( 'NONE', #127834, #27192, #35345, .T. ) ;
#13459=FACE_OUTER_BOUND ( 'NONE', #81914, .T. ) ;
#13460=DIRECTION ( 'NONE',  ( 0.000000000000000000, 1.000000000000000000, 0.000000000000000000 ) ) ;
#13461=ORIENTED_EDGE ( 'NONE', *, *, #112359, .T. ) ;
#13462=CARTESIAN_POINT ( 'NONE',  ( -11.05000000000000071, 2.500000000000000000, -2.611473670974873595 ) ) ;
#13463=DIRECTION ( 'NONE',  ( 0.000000000000000000, 0.000000000000000000, -1.000000000000000000 ) ) ;
#13464=ORIENTED_EDGE ( 'NONE', *, *, #110622, .F. ) ;
#13465=EDGE_CURVE ( 'NONE', #85004, #82670, #33207, .T. ) ;
#13466=CIRCLE ( 'NONE', #124298, 0.06509327318403745899 ) ;
#13467=ORIENTED_EDGE ( 'NONE', *, *, #91212, .F. ) ;
#13468=FACE_OUTER_BOUND ( 'NONE', #88251, .T. ) ;
#13470=ORIENTED_EDGE ( 'NONE', *, *, #32295, .F. ) ;
#13471=CARTESIAN_POINT ( 'NONE',  ( 0.1999999999999567124, 2.500000000000000000, -3.983716857408426293 ) ) ;
#13472=ORIENTED_EDGE ( 'NONE', *, *, #24198, .F. ) ;
#13473=CARTESIAN_POINT ( 'NONE',  ( -6.900000000000019007, 12.50000000000000000, -4.611443907251940644 ) ) ;
#13474=CARTESIAN_POINT ( 'NONE',  ( -8.950000000000011724, 12.50000000000000000, -6.083687093685483660 ) ) ;
#13475=AXIS2_PLACEMENT_3D ( 'NONE', #71825, #23340, #63283 ) ;
#13476=DIRECTION ( 'NONE',  ( -0.000000000000000000, 1.000000000000000000, -0.000000000000000000 ) ) ;
#13478=ORIENTED_EDGE ( 'NONE', *, *, #30809, .F. ) ;
#13479=FACE_OUTER_BOUND ( 'NONE', #81303, .T. ) ;
#13480=VERTEX_POINT ( 'NONE', #93024 ) ;
#13481=DIRECTION ( 'NONE',  ( -0.000000000000000000, 1.000000000000000000, -0.000000000000000000 ) ) ;
#13482=LINE ( 'NONE', #101237, #6925 ) ;
#13483=ORIENTED_EDGE ( 'NONE', *, *, #9053, .F. ) ;
#13484=CONICAL_SURFACE ( 'NONE', #55278, 0.1000000000000002554, 0.003490658503988666988 ) ;
#13486=ORIENTED_EDGE ( 'NONE', *, *, #60242, .T. ) ;
#13487=CIRCLE ( 'NONE', #63694, 0.1000000000000002554 ) ;
#13488=EDGE_LOOP ( 'NONE', ( #86289, #118077, #98582, #30780 ) ) ;
#13489=EDGE_LOOP ( 'NONE', ( #58015, #18694 ) ) ;
#13490=DIRECTION ( 'NONE',  ( 0.000000000000000000, 0.000000000000000000, 1.000000000000000000 ) ) ;
#13491=CARTESIAN_POINT ( 'NONE',  ( 5.399999999999932854, 2.500000000000000000, 3.637306695894644726 ) ) ;
#13492=CARTESIAN_POINT ( 'NONE',  ( 2.299999999999946976, 2.500000000000000000, 4.676537180435972552 ) ) ;
#13493=EDGE_CURVE ( 'NONE', #15344, #91497, #66626, .T. ) ;
#13494=FACE_BOUND ( 'NONE', #15515, .T. ) ;
#13495=ORIENTED_EDGE ( 'NONE', *, *, #59152, .T. ) ;
#13497=EDGE_CURVE ( 'NONE', #55738, #101182, #121014, .T. ) ;
#13498=DIRECTION ( 'NONE',  ( 0.000000000000000000, 1.000000000000000000, 0.000000000000000000 ) ) ;
#13499=LINE ( 'NONE', #24630, #12531 ) ;
#13500=AXIS2_PLACEMENT_3D ( 'NONE', #74390, #4329, #44277 ) ;
#13501=ADVANCED_FACE ( 'NONE', ( #45856 ), #106347, .T. ) ;
#13503=EDGE_CURVE ( 'NONE', #64922, #17072, #114742, .T. ) ;
#13504=CARTESIAN_POINT ( 'NONE',  ( 12.49999999999990585, 2.500000000000000000, -5.022947341949754119 ) ) ;
#13505=VECTOR ( 'NONE', #86458, 1000.000000000000000 ) ;
#13506=EDGE_CURVE ( 'NONE', #20279, #9507, #22744, .T. ) ;
#13508=CONICAL_SURFACE ( 'NONE', #34468, 0.1000000000000000472, 0.003490658503988666988 ) ;
#13509=CARTESIAN_POINT ( 'NONE',  ( -3.750000000000027534, 2.500000000000000000, -1.472243186433550122 ) ) ;
#13510=EDGE_CURVE ( 'NONE', #113395, #5884, #68778, .T. ) ;
#13511=EDGE_LOOP ( 'NONE', ( #89884, #75266 ) ) ;
#13512=EDGE_LOOP ( 'NONE', ( #70620, #69584, #105066, #11918 ) ) ;
#13513=ORIENTED_EDGE ( 'NONE', *, *, #122854, .T. ) ;
#13514=VERTEX_POINT ( 'NONE', #106058 ) ;
#13515=ORIENTED_EDGE ( 'NONE', *, *, #105325, .T. ) ;
#13517=DIRECTION ( 'NONE',  ( -0.000000000000000000, -1.000000000000000000, -0.000000000000000000 ) ) ;
#13518=EDGE_LOOP ( 'NONE', ( #95037, #80468, #118525, #112893 ) ) ;
#13519=FACE_BOUND ( 'NONE', #63268, .T. ) ;
#13520=EDGE_CURVE ( 'NONE', #40491, #3245, #26929, .T. ) ;
#13521=CARTESIAN_POINT ( 'NONE',  ( -6.450000000000019718, 2.500000000000000000, -6.048780366869526581 ) ) ;
#13522=CONICAL_SURFACE ( 'NONE', #80448, 0.1000000000000002554, 0.003490658503988666988 ) ;
#13523=VECTOR ( 'NONE', #93954, 1000.000000000000000 ) ;
#13524=VECTOR ( 'NONE', #46120, 1000.000000000000000 ) ;
#13526=AXIS2_PLACEMENT_3D ( 'NONE', #95343, #23356, #33834 ) ;
#13527=DIRECTION ( 'NONE',  ( 0.000000000000000000, -0.9999939076577903929, 0.003490651415223739937 ) ) ;
#13528=DIRECTION ( 'NONE',  ( 1.000000000000000000, 0.000000000000000000, 0.000000000000000000 ) ) ;
#13530=ORIENTED_EDGE ( 'NONE', *, *, #73504, .F. ) ;
#13532=CONICAL_SURFACE ( 'NONE', #82604, 0.1000000000000000056, 0.003490658503988666988 ) ;
#13533=VERTEX_POINT ( 'NONE', #126992 ) ;
#13534=AXIS2_PLACEMENT_3D ( 'NONE', #91847, #51928, #2814 ) ;
#13535=ORIENTED_EDGE ( 'NONE', *, *, #65057, .F. ) ;
#13536=ORIENTED_EDGE ( 'NONE', *, *, #47499, .T. ) ;
#13537=DIRECTION ( 'NONE',  ( 0.000000000000000000, 1.000000000000000000, 0.000000000000000000 ) ) ;
#13538=VECTOR ( 'NONE', #122948, 1000.000000000000000 ) ;
#13539=DIRECTION ( 'NONE',  ( -0.000000000000000000, 1.000000000000000000, -0.000000000000000000 ) ) ;
#13540=DIRECTION ( 'NONE',  ( 0.000000000000000000, -0.000000000000000000, 1.000000000000000000 ) ) ;
#13541=ORIENTED_EDGE ( 'NONE', *, *, #49552, .F. ) ;
#13542=DIRECTION ( 'NONE',  ( 0.000000000000000000, 0.000000000000000000, 1.000000000000000000 ) ) ;
#13543=CIRCLE ( 'NONE', #44959, 0.1000000000000002554 ) ;
#13544=CIRCLE ( 'NONE', #30212, 0.06509327318403743123 ) ;
#13545=DIRECTION ( 'NONE',  ( 0.000000000000000000, -0.000000000000000000, 1.000000000000000000 ) ) ;
#13546=CARTESIAN_POINT ( 'NONE',  ( -3.749999999999991118, 2.500000000000000000, 2.165063509461097713 ) ) ;
#13548=ORIENTED_EDGE ( 'NONE', *, *, #110064, .T. ) ;
#13549=DIRECTION ( 'NONE',  ( 0.000000000000000000, 0.000000000000000000, 1.000000000000000000 ) ) ;
#13550=EDGE_LOOP ( 'NONE', ( #120272, #103018, #85423, #115243 ) ) ;
#13552=ORIENTED_EDGE ( 'NONE', *, *, #122864, .F. ) ;
#13553=EDGE_CURVE ( 'NONE', #119152, #86156, #16986, .T. ) ;
#13554=ORIENTED_EDGE ( 'NONE', *, *, #105431, .F. ) ;
#13555=LINE ( 'NONE', #24044, #70155 ) ;
#13556=CARTESIAN_POINT ( 'NONE',  ( 10.84999999999990905, 2.500000000000000000, -5.902370205355750521 ) ) ;
#13557=PLANE ( 'NONE',  #50904 ) ;
#13558=DIRECTION ( 'NONE',  ( 0.000000000000000000, 0.000000000000000000, 1.000000000000000000 ) ) ;
#13559=LINE ( 'NONE', #53509, #43447 ) ;
#13561=ORIENTED_EDGE ( 'NONE', *, *, #66420, .F. ) ;
#13562=VERTEX_POINT ( 'NONE', #18311 ) ;
#13563=EDGE_CURVE ( 'NONE', #33691, #120278, #49935, .T. ) ;
#13564=CARTESIAN_POINT ( 'NONE',  ( 0.3999999999999559464, 12.50000000000000000, -4.330127018922201643 ) ) ;
#13565=DIRECTION ( 'NONE',  ( 0.000000000000000000, 1.000000000000000000, 0.000000000000000000 ) ) ;
#13566=CARTESIAN_POINT ( 'NONE',  ( -0.6000000000000388356, 2.500000000000000000, 3.983716857408420964 ) ) ;
#13567=EDGE_LOOP ( 'NONE', ( #121236, #27837 ) ) ;
#13568=VERTEX_POINT ( 'NONE', #57611 ) ;
#13569=DIRECTION ( 'NONE',  ( 0.000000000000000000, 0.000000000000000000, 1.000000000000000000 ) ) ;
#13570=CIRCLE ( 'NONE', #26199, 0.06509327318403745899 ) ;
#13571=EDGE_LOOP ( 'NONE', ( #65108, #43647 ) ) ;
#13572=CARTESIAN_POINT ( 'NONE',  ( 2.899999999999944844, 12.50000000000000000, 3.637306695894644726 ) ) ;
#13573=CIRCLE ( 'NONE', #105534, 0.09999999999999982514 ) ;
#13574=CARTESIAN_POINT ( 'NONE',  ( 4.599999999999938360, 2.500000000000000000, -0.5928203230275541635 ) ) ;
#13575=EDGE_LOOP ( 'NONE', ( #5209, #109289 ) ) ;
#13576=CARTESIAN_POINT ( 'NONE',  ( -5.400000000000023448, 12.50000000000000000, -5.022947341949754119 ) ) ;
#13577=DIRECTION ( 'NONE',  ( -0.000000000000000000, 1.000000000000000000, -0.000000000000000000 ) ) ;
#13578=DIRECTION ( 'NONE',  ( 0.000000000000000000, 0.000000000000000000, 1.000000000000000000 ) ) ;
#13579=LINE ( 'NONE', #3139, #84464 ) ;
#13580=CARTESIAN_POINT ( 'NONE',  ( -7.900000000000014566, 2.500000000000000000, -4.430127018922202176 ) ) ;
#13581=ORIENTED_EDGE ( 'NONE', *, *, #33478, .T. ) ;
#13582=CIRCLE ( 'NONE', #88809, 0.1000000000000002554 ) ;
#13583=DIRECTION ( 'NONE',  ( -0.000000000000000000, 1.000000000000000000, -0.000000000000000000 ) ) ;
#13584=CARTESIAN_POINT ( 'NONE',  ( -9.350000000000004974, 2.500000000000000000, 6.148780366869520897 ) ) ;
#13585=AXIS2_PLACEMENT_3D ( 'NONE', #6416, #14321, #66649 ) ;
#13586=ORIENTED_EDGE ( 'NONE', *, *, #30883, .T. ) ;
#13587=ORIENTED_EDGE ( 'NONE', *, *, #127280, .F. ) ;
#13589=CARTESIAN_POINT ( 'NONE',  ( -7.950000000000009059, 2.500000000000000000, 6.495190528383297135 ) ) ;
#13590=CARTESIAN_POINT ( 'NONE',  ( -10.85000000000000142, 12.50000000000000000, -5.802370205355746435 ) ) ;
#13591=FACE_OUTER_BOUND ( 'NONE', #3589, .T. ) ;
#13592=CARTESIAN_POINT ( 'NONE',  ( -4.600000000000024514, 12.50000000000000000, 0.6928203230275494784 ) ) ;
#13593=ADVANCED_FACE ( 'NONE', ( #16360 ), #129362, .T. ) ;
#13594=CIRCLE ( 'NONE', #36617, 0.06509327318403745899 ) ;
#13595=CARTESIAN_POINT ( 'NONE',  ( -1.850000000000033840, 12.50000000000000000, 6.213873640053559022 ) ) ;
#13596=AXIS2_PLACEMENT_3D ( 'NONE', #52660, #53324, #41583 ) ;
#13597=CARTESIAN_POINT ( 'NONE',  ( 1.699999999999950218, 2.500000000000000000, 4.330127018922196314 ) ) ;
#13598=DIRECTION ( 'NONE',  ( -0.000000000000000000, 1.000000000000000000, -0.000000000000000000 ) ) ;
#13599=DIRECTION ( 'NONE',  ( 0.000000000000000000, 0.000000000000000000, 1.000000000000000000 ) ) ;
#13602=EDGE_CURVE ( 'NONE', #98295, #41903, #56159, .T. ) ;
#13603=ORIENTED_EDGE ( 'NONE', *, *, #67377, .F. ) ;
#13604=ORIENTED_EDGE ( 'NONE', *, *, #100409, .T. ) ;
#13605=EDGE_LOOP ( 'NONE', ( #43808, #122746, #113392, #75983 ) ) ;
#13606=ADVANCED_FACE ( 'NONE', ( #97518 ), #28147, .T. ) ;
#13607=ORIENTED_EDGE ( 'NONE', *, *, #87358, .F. ) ;
#13608=EDGE_CURVE ( 'NONE', #71950, #12555, #54115, .T. ) ;
#13609=CONICAL_SURFACE ( 'NONE', #51305, 0.1000000000000000472, 0.003490658503988666988 ) ;
#13610=CARTESIAN_POINT ( 'NONE',  ( 11.89999999999990798, 2.500000000000000000, -4.083716857408426826 ) ) ;
#13611=DIRECTION ( 'NONE',  ( 0.000000000000000000, 0.000000000000000000, 1.000000000000000000 ) ) ;
#13612=VERTEX_POINT ( 'NONE', #116512 ) ;
#13613=CARTESIAN_POINT ( 'NONE',  ( 3.099999999999944134, 2.500000000000000000, 4.676537180435972552 ) ) ;
#13614=CIRCLE ( 'NONE', #86776, 0.1000000000000000472 ) ;
#13615=EDGE_CURVE ( 'NONE', #31532, #42779, #127289, .T. ) ;
#13616=VECTOR ( 'NONE', #35050, 1000.000000000000000 ) ;
#13617=DIRECTION ( 'NONE',  ( 0.000000000000000000, -0.000000000000000000, 1.000000000000000000 ) ) ;
#13618=CARTESIAN_POINT ( 'NONE',  ( 5.449999999999934452, 12.50000000000000000, 2.165063509461097713 ) ) ;
#13619=ORIENTED_EDGE ( 'NONE', *, *, #36993, .F. ) ;
#13620=CIRCLE ( 'NONE', #101467, 0.1000000000000002554 ) ;
#13621=EDGE_CURVE ( 'NONE', #73563, #74488, #39475, .T. ) ;
#13622=LINE ( 'NONE', #64663, #18189 ) ;
#13624=VERTEX_POINT ( 'NONE', #68705 ) ;
#13625=VECTOR ( 'NONE', #76065, 1000.000000000000000 ) ;
#13626=CONICAL_SURFACE ( 'NONE', #30389, 0.1000000000000002554, 0.003490658503988666988 ) ;
#13627=ORIENTED_EDGE ( 'NONE', *, *, #123403, .T. ) ;
#13628=ORIENTED_EDGE ( 'NONE', *, *, #127435, .F. ) ;
#13629=EDGE_LOOP ( 'NONE', ( #115845, #34183, #91288, #118627 ) ) ;
#13630=DIRECTION ( 'NONE',  ( 0.000000000000000000, -0.9999939076577903929, 0.003490651415223739937 ) ) ;
#13631=DIRECTION ( 'NONE',  ( 0.000000000000000000, 1.000000000000000000, 0.000000000000000000 ) ) ;
#13632=CARTESIAN_POINT ( 'NONE',  ( 1.649999999999951061, 12.50000000000000000, -6.430097255199264339 ) ) ;
#13633=VECTOR ( 'NONE', #13439, 1000.000000000000000 ) ;
#13634=DIRECTION ( 'NONE',  ( 0.000000000000000000, 1.000000000000000000, 0.000000000000000000 ) ) ;
#13635=CIRCLE ( 'NONE', #80477, 0.1000000000000002554 ) ;
#13636=ORIENTED_EDGE ( 'NONE', *, *, #19931, .T. ) ;
#13637=FACE_OUTER_BOUND ( 'NONE', #84356, .T. ) ;
#13638=AXIS2_PLACEMENT_3D ( 'NONE', #118571, #66893, #79324 ) ;
#13639=VERTEX_POINT ( 'NONE', #46481 ) ;
#13640=CARTESIAN_POINT ( 'NONE',  ( -9.999999999999971578, 2.500000000000000000, -4.330127018922197202 ) ) ;
#13641=DIRECTION ( 'NONE',  ( -0.000000000000000000, 1.000000000000000000, -0.000000000000000000 ) ) ;
#13642=CARTESIAN_POINT ( 'NONE',  ( 12.49999999999990408, 12.50000000000000000, -3.637306695894650055 ) ) ;
#13643=CARTESIAN_POINT ( 'NONE',  ( 4.149999999999936406, 2.500000000000000000, 6.495190528383297135 ) ) ;
#13644=ORIENTED_EDGE ( 'NONE', *, *, #119407, .T. ) ;
#13645=ORIENTED_EDGE ( 'NONE', *, *, #2111, .F. ) ;
#13647=DIRECTION ( 'NONE',  ( -0.000000000000000000, 1.000000000000000000, -0.000000000000000000 ) ) ;
#13648=DIRECTION ( 'NONE',  ( 0.000000000000000000, 1.000000000000000000, 0.000000000000000000 ) ) ;
#13649=DIRECTION ( 'NONE',  ( 0.000000000000000000, 0.000000000000000000, -1.000000000000000000 ) ) ;
#13650=FACE_BOUND ( 'NONE', #91976, .T. ) ;
#13651=CARTESIAN_POINT ( 'NONE',  ( -8.150000000000014566, 12.50000000000000000, -6.841600689897073373 ) ) ;
#13652=CIRCLE ( 'NONE', #97289, 0.06509327318403745899 ) ;
#13653=DIRECTION ( 'NONE',  ( 0.000000000000000000, 0.000000000000000000, -1.000000000000000000 ) ) ;
#13654=ADVANCED_FACE ( 'NONE', ( #106690 ), #115874, .T. ) ;
#13655=CARTESIAN_POINT ( 'NONE',  ( 8.549999999999918998, 12.50000000000000000, 6.841600689897072485 ) ) ;
#13656=EDGE_CURVE ( 'NONE', #21944, #98236, #123078, .T. ) ;
#13657=CARTESIAN_POINT ( 'NONE',  ( -2.500000000000032419, 2.500000000000000000, -3.537306695894649966 ) ) ;
#13658=AXIS2_PLACEMENT_3D ( 'NONE', #93091, #94352, #4662 ) ;
#13660=ADVANCED_FACE ( 'NONE', ( #78553 ), #8483, .T. ) ;
#13661=CARTESIAN_POINT ( 'NONE',  ( 3.099999999999945022, 2.500000000000000000, -4.676537180435978769 ) ) ;
#13662=VERTEX_POINT ( 'NONE', #58900 ) ;
#13663=CIRCLE ( 'NONE', #118317, 0.1000000000000002554 ) ;
#13664=EDGE_CURVE ( 'NONE', #85870, #74320, #98805, .T. ) ;
#13665=AXIS2_PLACEMENT_3D ( 'NONE', #95945, #6253, #46197 ) ;
#13666=PLANE ( 'NONE',  #1488 ) ;
#13667=EDGE_CURVE ( 'NONE', #102762, #120000, #116799, .T. ) ;
#13668=EDGE_LOOP ( 'NONE', ( #6709, #88019, #87302, #120981 ) ) ;
#13669=EDGE_LOOP ( 'NONE', ( #99546, #128770 ) ) ;
#13670=ORIENTED_EDGE ( 'NONE', *, *, #9910, .F. ) ;
#13671=CARTESIAN_POINT ( 'NONE',  ( -12.69999999999999396, 2.500000000000000000, 0.3464101615137776813 ) ) ;
#13672=FACE_BOUND ( 'NONE', #55416, .T. ) ;
#13673=FACE_OUTER_BOUND ( 'NONE', #84866, .T. ) ;
#13674=EDGE_CURVE ( 'NONE', #121706, #78315, #100094, .T. ) ;
#13675=CONICAL_SURFACE ( 'NONE', #49219, 0.1000000000000000472, 0.003490658503988666988 ) ;
#13676=EDGE_CURVE ( 'NONE', #114100, #52047, #62447, .T. ) ;
#13677=CIRCLE ( 'NONE', #65913, 0.09999999999999982514 ) ;
#13678=ORIENTED_EDGE ( 'NONE', *, *, #20758, .T. ) ;
#13679=DIRECTION ( 'NONE',  ( 0.000000000000000000, 0.000000000000000000, 1.000000000000000000 ) ) ;
#13680=DIRECTION ( 'NONE',  ( 0.000000000000000000, 0.000000000000000000, 1.000000000000000000 ) ) ;
#13682=DIRECTION ( 'NONE',  ( 0.000000000000000000, -0.9999939076577903929, 0.003490651415223739937 ) ) ;
#13683=DIRECTION ( 'NONE',  ( -0.000000000000000000, -1.000000000000000000, -0.000000000000000000 ) ) ;
#13684=AXIS2_PLACEMENT_3D ( 'NONE', #8667, #49934, #120584 ) ;
#13685=AXIS2_PLACEMENT_3D ( 'NONE', #79407, #7413, #87900 ) ;
#13686=B_SPLINE_CURVE_WITH_KNOTS ( 'NONE', 3,
 ( #84688, #44123, #95799, #5467, #93233, #95161, #6116, #15930, #103699, #116082 ),
 .UNSPECIFIED., .F., .F.,
 ( 4, 2, 2, 2, 4 ),
 ( 0.003751885956794874175, 0.02035553200375761485, 0.03695917805072035378, 0.05356282409768309272, 0.07016647014464583165 ),
 .UNSPECIFIED. ) ;
#13687=EDGE_LOOP ( 'NONE', ( #61164, #7318 ) ) ;
#13688=DIRECTION ( 'NONE',  ( 0.000000000000000000, 0.000000000000000000, 1.000000000000000000 ) ) ;
#13689=CARTESIAN_POINT ( 'NONE',  ( -11.64999999999999680, 12.50000000000000000, 2.099970236277060032 ) ) ;
#13691=ORIENTED_EDGE ( 'NONE', *, *, #19671, .F. ) ;
#13692=CARTESIAN_POINT ( 'NONE',  ( -14.14999999999998792, 2.500000000000000000, -1.472243186433547901 ) ) ;
#13693=DIRECTION ( 'NONE',  ( -4.274815082592931898E-19, -0.9999939076577903929, -0.003490651415223739937 ) ) ;
#13694=CONICAL_SURFACE ( 'NONE', #26239, 0.1000000000000002554, 0.003490658503988666988 ) ;
#13695=DIRECTION ( 'NONE',  ( 0.000000000000000000, 1.000000000000000000, 0.000000000000000000 ) ) ;
#13696=ORIENTED_EDGE ( 'NONE', *, *, #117371, .T. ) ;
#13697=ORIENTED_EDGE ( 'NONE', *, *, #92558, .F. ) ;
#13698=EDGE_CURVE ( 'NONE', #127947, #102323, #64571, .T. ) ;
#13699=CARTESIAN_POINT ( 'NONE',  ( 4.799999999999937650, 2.500000000000000000, -0.4464101615137782142 ) ) ;
#13700=AXIS2_PLACEMENT_3D ( 'NONE', #50957, #62066, #80413 ) ;
#13701=ORIENTED_EDGE ( 'NONE', *, *, #109733, .T. ) ;
#13702=CARTESIAN_POINT ( 'NONE',  ( 0.6499999999999561684, 12.50000000000000000, -1.818653347947325916 ) ) ;
#13703=FACE_OUTER_BOUND ( 'NONE', #21415, .T. ) ;
#13704=VERTEX_POINT ( 'NONE', #112982 ) ;
#13705=CIRCLE ( 'NONE', #32525, 0.06509327318403745899 ) ;
#13706=DIRECTION ( 'NONE',  ( 0.000000000000000000, 1.000000000000000000, 0.000000000000000000 ) ) ;
#13707=DIRECTION ( 'NONE',  ( -0.000000000000000000, 1.000000000000000000, -0.000000000000000000 ) ) ;
#13708=FACE_OUTER_BOUND ( 'NONE', #79972, .T. ) ;
#13710=CARTESIAN_POINT ( 'NONE',  ( -10.45000000000000107, 2.500000000000000000, 6.395190528383296602 ) ) ;
#13711=AXIS2_PLACEMENT_3D ( 'NONE', #34874, #63678, #74781 ) ;
#13712=EDGE_LOOP ( 'NONE', ( #111843, #60130 ) ) ;
#13714=EDGE_LOOP ( 'NONE', ( #116360, #29678 ) ) ;
#13715=CARTESIAN_POINT ( 'NONE',  ( -4.600000000000025402, 12.50000000000000000, 4.330127018922196314 ) ) ;
#13716=DIRECTION ( 'NONE',  ( 0.000000000000000000, 0.000000000000000000, 1.000000000000000000 ) ) ;
#13717=CONICAL_SURFACE ( 'NONE', #11676, 0.1000000000000002554, 0.003490658503988666988 ) ;
#13718=ORIENTED_EDGE ( 'NONE', *, *, #29086, .T. ) ;
#13719=ORIENTED_EDGE ( 'NONE', *, *, #26864, .F. ) ;
#13721=DIRECTION ( 'NONE',  ( 0.000000000000000000, 1.000000000000000000, 0.000000000000000000 ) ) ;
#13722=CONICAL_SURFACE ( 'NONE', #17939, 0.09999999999999982514, 0.003490658503988666988 ) ;
#13723=DIRECTION ( 'NONE',  ( 0.000000000000000000, -0.9999939076577903929, 0.003490651415223739937 ) ) ;
#13724=VECTOR ( 'NONE', #119305, 1000.000000000000000 ) ;
#13725=CARTESIAN_POINT ( 'NONE',  ( -13.34999999999999076, 2.500000000000000000, 2.165063509461101265 ) ) ;
#13726=AXIS2_PLACEMENT_3D ( 'NONE', #78796, #108862, #118692 ) ;
#13728=CARTESIAN_POINT ( 'NONE',  ( -12.69999999999999218, 2.500000000000000000, -0.4464101615137741064 ) ) ;
#13730=DIRECTION ( 'NONE',  ( 0.000000000000000000, -0.000000000000000000, 1.000000000000000000 ) ) ;
#13731=CIRCLE ( 'NONE', #43023, 0.06509327318403745899 ) ;
#13732=FACE_OUTER_BOUND ( 'NONE', #92275, .T. ) ;
#13733=CARTESIAN_POINT ( 'NONE',  ( -7.900000000000011013, 2.500000000000000000, 3.537306695894645081 ) ) ;
#13734=PLANE ( 'NONE',  #56117 ) ;
#13735=VERTEX_POINT ( 'NONE', #69340 ) ;
#13736=DIRECTION ( 'NONE',  ( 0.000000000000000000, 0.000000000000000000, 1.000000000000000000 ) ) ;
#13737=ORIENTED_EDGE ( 'NONE', *, *, #51079, .F. ) ;
#13738=ORIENTED_EDGE ( 'NONE', *, *, #81915, .T. ) ;
#13739=CARTESIAN_POINT ( 'NONE',  ( -8.950000000000009948, 12.50000000000000000, -1.818653347947326138 ) ) ;
#13740=DIRECTION ( 'NONE',  ( -0.000000000000000000, 1.000000000000000000, -0.000000000000000000 ) ) ;
#13741=CONICAL_SURFACE ( 'NONE', #61894, 0.1000000000000000056, 0.003490658503988666988 ) ;
#13743=DIRECTION ( 'NONE',  ( 0.000000000000000000, 0.000000000000000000, 1.000000000000000000 ) ) ;
#13745=DIRECTION ( 'NONE',  ( 0.000000000000000000, 0.000000000000000000, 1.000000000000000000 ) ) ;
#13747=CARTESIAN_POINT ( 'NONE',  ( 11.24999999999994316, 2.500000000000000000, 2.165063509461097713 ) ) ;
#13748=ORIENTED_EDGE ( 'NONE', *, *, #54287, .T. ) ;
#13749=DIRECTION ( 'NONE',  ( 0.000000000000000000, 0.000000000000000000, -1.000000000000000000 ) ) ;
#13750=AXIS2_PLACEMENT_3D ( 'NONE', #48485, #98218, #58322 ) ;
#13751=CIRCLE ( 'NONE', #78636, 0.1000000000000002554 ) ;
#13752=CIRCLE ( 'NONE', #101604, 0.1000000000000002554 ) ;
#13753=CARTESIAN_POINT ( 'NONE',  ( -6.850000000000017408, 2.500000000000000000, -2.511473670974877948 ) ) ;
#13754=ORIENTED_EDGE ( 'NONE', *, *, #70109, .F. ) ;
#13755=EDGE_CURVE ( 'NONE', #28046, #11893, #129594, .T. ) ;
#13756=ORIENTED_EDGE ( 'NONE', *, *, #81773, .T. ) ;
#13757=AXIS2_PLACEMENT_3D ( 'NONE', #98195, #87721, #36062 ) ;
#13758=ORIENTED_EDGE ( 'NONE', *, *, #34230, .T. ) ;
#13759=ADVANCED_FACE ( 'NONE', ( #62609 ), #39913, .T. ) ;
#13760=VERTEX_POINT ( 'NONE', #3673 ) ;
#13762=DIRECTION ( 'NONE',  ( -0.000000000000000000, -1.000000000000000000, -0.000000000000000000 ) ) ;
#13763=FACE_OUTER_BOUND ( 'NONE', #99855, .T. ) ;
#13764=AXIS2_PLACEMENT_3D ( 'NONE', #80494, #68711, #108638 ) ;
#13765=DIRECTION ( 'NONE',  ( 0.000000000000000000, -0.9999939076577903929, 0.003490651415223739937 ) ) ;
#13766=LINE ( 'NONE', #53704, #4741 ) ;
#13767=AXIS2_PLACEMENT_3D ( 'NONE', #125601, #47073, #27395 ) ;
#13768=CIRCLE ( 'NONE', #91152, 0.1000000000000002554 ) ;
#13769=EDGE_CURVE ( 'NONE', #88360, #17776, #45810, .T. ) ;
#13770=DIRECTION ( 'NONE',  ( 0.000000000000000000, 0.000000000000000000, 1.000000000000000000 ) ) ;
#13771=ADVANCED_FACE ( 'NONE', ( #30099 ), #116880, .T. ) ;
#13772=ORIENTED_EDGE ( 'NONE', *, *, #108457, .T. ) ;
#13773=DIRECTION ( 'NONE',  ( -0.000000000000000000, -1.000000000000000000, -0.000000000000000000 ) ) ;
#13774=EDGE_CURVE ( 'NONE', #74262, #46085, #52770, .T. ) ;
#13775=DIRECTION ( 'NONE',  ( 0.000000000000000000, 1.000000000000000000, 0.000000000000000000 ) ) ;
#13776=EDGE_CURVE ( 'NONE', #57128, #103454, #119736, .T. ) ;
#13777=CARTESIAN_POINT ( 'NONE',  ( -12.49999999999999289, 2.500000000000000000, -5.122947341949751987 ) ) ;
#13778=DIRECTION ( 'NONE',  ( -0.000000000000000000, -1.000000000000000000, -0.000000000000000000 ) ) ;
#13779=EDGE_LOOP ( 'NONE', ( #108950, #115453, #30838, #23655 ) ) ;
#13780=VERTEX_POINT ( 'NONE', #109937 ) ;
#13781=ORIENTED_EDGE ( 'NONE', *, *, #107633, .F. ) ;
#13782=FACE_OUTER_BOUND ( 'NONE', #103297, .T. ) ;
#13783=EDGE_CURVE ( 'NONE', #83794, #65306, #89710, .T. ) ;
#13784=CARTESIAN_POINT ( 'NONE',  ( 2.899999999999946620, 2.500000000000000000, -3.537306695894649966 ) ) ;
#13785=CARTESIAN_POINT ( 'NONE',  ( -11.24999999999996270, 2.500000000000000000, 2.165063509461097713 ) ) ;
#13786=ORIENTED_EDGE ( 'NONE', *, *, #33497, .F. ) ;
#13787=LINE ( 'NONE', #102809, #85007 ) ;
#13788=DIRECTION ( 'NONE',  ( 0.000000000000000000, 0.000000000000000000, 1.000000000000000000 ) ) ;
#13789=DIRECTION ( 'NONE',  ( -4.274815082592931898E-19, -0.9999939076577903929, -0.003490651415223739937 ) ) ;
#13790=CARTESIAN_POINT ( 'NONE',  ( -0.8500000000000386136, 2.500000000000000000, 5.902370205355745192 ) ) ;
#13791=AXIS2_PLACEMENT_3D ( 'NONE', #17731, #17062, #57011 ) ;
#13792=CARTESIAN_POINT ( 'NONE',  ( -1.650000000000034328, 12.50000000000000000, -6.495190528383302464 ) ) ;
#13793=VECTOR ( 'NONE', #45196, 1000.000000000000000 ) ;
#13794=ORIENTED_EDGE ( 'NONE', *, *, #56774, .T. ) ;
#13795=EDGE_LOOP ( 'NONE', ( #50717, #19584 ) ) ;
#13798=DIRECTION ( 'NONE',  ( 0.000000000000000000, 0.000000000000000000, -1.000000000000000000 ) ) ;
#13799=LINE ( 'NONE', #113298, #47055 ) ;
#13800=DIRECTION ( 'NONE',  ( 0.000000000000000000, -0.000000000000000000, 1.000000000000000000 ) ) ;
#13801=AXIS2_PLACEMENT_3D ( 'NONE', #126210, #8999, #106558 ) ;
#13802=FACE_OUTER_BOUND ( 'NONE', #109017, .T. ) ;
#13803=ORIENTED_EDGE ( 'NONE', *, *, #15112, .T. ) ;
#13804=EDGE_CURVE ( 'NONE', #24108, #124192, #23966, .T. ) ;
#13805=ORIENTED_EDGE ( 'NONE', *, *, #39599, .F. ) ;
#13806=ADVANCED_FACE ( 'NONE', ( #79194 ), #9788, .T. ) ;
#13807=DIRECTION ( 'NONE',  ( 0.000000000000000000, -0.000000000000000000, 1.000000000000000000 ) ) ;
#13808=CARTESIAN_POINT ( 'NONE',  ( -7.100000000000017408, 2.500000000000000000, -3.737306695894649700 ) ) ;
#13809=DIRECTION ( 'NONE',  ( 0.000000000000000000, 1.000000000000000000, 0.000000000000000000 ) ) ;
#13810=EDGE_CURVE ( 'NONE', #72978, #125967, #43765, .T. ) ;
#13813=CONICAL_SURFACE ( 'NONE', #105865, 0.09999999999999982514, 0.003490658503988666988 ) ;
#13814=DIRECTION ( 'NONE',  ( -4.274815082592931898E-19, -0.9999939076577903929, -0.003490651415223739937 ) ) ;
#13815=EDGE_CURVE ( 'NONE', #57879, #22979, #84806, .T. ) ;
#13816=VECTOR ( 'NONE', #40656, 1000.000000000000000 ) ;
#13818=EDGE_CURVE ( 'NONE', #122473, #77164, #123167, .T. ) ;
#13819=ORIENTED_EDGE ( 'NONE', *, *, #23379, .F. ) ;
#13820=FACE_OUTER_BOUND ( 'NONE', #112830, .T. ) ;
#13821=EDGE_CURVE ( 'NONE', #10798, #73823, #114268, .T. ) ;
#13822=ORIENTED_EDGE ( 'NONE', *, *, #36976, .T. ) ;
#13823=DIRECTION ( 'NONE',  ( 0.000000000000000000, 1.000000000000000000, 0.000000000000000000 ) ) ;
#13824=EDGE_CURVE ( 'NONE', #12959, #113477, #26543, .T. ) ;
#13825=EDGE_CURVE ( 'NONE', #69331, #17546, #22836, .T. ) ;
#13826=EDGE_CURVE ( 'NONE', #87887, #19796, #100182, .T. ) ;
#13827=ORIENTED_EDGE ( 'NONE', *, *, #27127, .F. ) ;
#13828=CARTESIAN_POINT ( 'NONE',  ( 4.599999999999936584, 2.500000000000000000, 3.637306695894644726 ) ) ;
#13829=CARTESIAN_POINT ( 'NONE',  ( -1.250000000000035749, 2.500000000000000000, -7.088010851410853519 ) ) ;
#13830=ORIENTED_EDGE ( 'NONE', *, *, #112679, .T. ) ;
#13831=VERTEX_POINT ( 'NONE', #124090 ) ;
#13833=CARTESIAN_POINT ( 'NONE',  ( -4.550000000000022915, 2.500000000000000000, 6.495190528383297135 ) ) ;
#13835=ADVANCED_FACE ( 'NONE', ( #95920 ), #95971, .T. ) ;
#13838=AXIS2_PLACEMENT_3D ( 'NONE', #12772, #33719, #113575 ) ;
#13839=DIRECTION ( 'NONE',  ( -0.000000000000000000, -1.000000000000000000, -0.000000000000000000 ) ) ;
#13840=CARTESIAN_POINT ( 'NONE',  ( 3.549999999999944755, 12.50000000000000000, -6.841600689897077814 ) ) ;
#13841=DIRECTION ( 'NONE',  ( 0.000000000000000000, 1.000000000000000000, 0.000000000000000000 ) ) ;
#13843=DIRECTION ( 'NONE',  ( -4.274815082592931898E-19, -0.9999939076577903929, -0.003490651415223739937 ) ) ;
#13844=CIRCLE ( 'NONE', #20123, 0.09999999999999982514 ) ;
#13845=AXIS2_PLACEMENT_3D ( 'NONE', #81939, #91128, #149 ) ;
#13846=ORIENTED_EDGE ( 'NONE', *, *, #62106, .F. ) ;
#13847=AXIS2_PLACEMENT_3D ( 'NONE', #54259, #33978, #73895 ) ;
#13848=VERTEX_POINT ( 'NONE', #4947 ) ;
#13849=DIRECTION ( 'NONE',  ( 0.000000000000000000, 0.000000000000000000, 1.000000000000000000 ) ) ;
#13850=ORIENTED_EDGE ( 'NONE', *, *, #61674, .F. ) ;
#13851=CARTESIAN_POINT ( 'NONE',  ( -12.09999999999999609, 2.500000000000000000, -3.637306695894647390 ) ) ;
#13852=FACE_OUTER_BOUND ( 'NONE', #64018, .T. ) ;
#13853=FACE_OUTER_BOUND ( 'NONE', #8807, .T. ) ;
#13854=ORIENTED_EDGE ( 'NONE', *, *, #91572, .F. ) ;
#13855=ORIENTED_EDGE ( 'NONE', *, *, #4207, .T. ) ;
#13856=DIRECTION ( 'NONE',  ( -4.274815082592931898E-19, -0.9999939076577903929, -0.003490651415223739937 ) ) ;
#13857=EDGE_LOOP ( 'NONE', ( #22699, #51731, #25820, #123209 ) ) ;
#13858=CARTESIAN_POINT ( 'NONE',  ( 11.44999999999990692, 2.500000000000000000, 1.818653347947321475 ) ) ;
#13859=DIRECTION ( 'NONE',  ( 0.000000000000000000, 0.000000000000000000, 1.000000000000000000 ) ) ;
#13860=AXIS2_PLACEMENT_3D ( 'NONE', #14917, #27330, #55533 ) ;
#13861=DIRECTION ( 'NONE',  ( -0.000000000000000000, -1.000000000000000000, -0.000000000000000000 ) ) ;
#13862=CARTESIAN_POINT ( 'NONE',  ( -13.09999999999999254, 12.50000000000000000, -4.676537180435975216 ) ) ;
#13863=CARTESIAN_POINT ( 'NONE',  ( 10.39999999999990976, 12.50000000000000000, 4.330127018922196314 ) ) ;
#13864=VECTOR ( 'NONE', #8408, 1000.000000000000000 ) ;
#13865=VECTOR ( 'NONE', #13046, 1000.000000000000000 ) ;
#13866=DIRECTION ( 'NONE',  ( 0.000000000000000000, 0.000000000000000000, 1.000000000000000000 ) ) ;
#13867=CARTESIAN_POINT ( 'NONE',  ( -5.400000000000019895, 2.500000000000000000, 4.330127018922196314 ) ) ;
#13870=DIRECTION ( 'NONE',  ( -0.000000000000000000, -1.000000000000000000, -0.000000000000000000 ) ) ;
#13871=CARTESIAN_POINT ( 'NONE',  ( 3.749999999999976907, 12.50000000000000000, 2.165063509461097713 ) ) ;
#13872=EDGE_LOOP ( 'NONE', ( #63528, #49035 ) ) ;
#13873=VERTEX_POINT ( 'NONE', #45547 ) ;
#13874=EDGE_CURVE ( 'NONE', #94218, #83042, #106381, .T. ) ;
#13875=ORIENTED_EDGE ( 'NONE', *, *, #104846, .F. ) ;
#13877=ORIENTED_EDGE ( 'NONE', *, *, #118017, .F. ) ;
#13878=DIRECTION ( 'NONE',  ( 0.000000000000000000, 0.000000000000000000, 1.000000000000000000 ) ) ;
#13879=ORIENTED_EDGE ( 'NONE', *, *, #51485, .T. ) ;
#13880=ORIENTED_EDGE ( 'NONE', *, *, #36285, .T. ) ;
#13881=EDGE_LOOP ( 'NONE', ( #50627, #121778, #11457, #127616 ) ) ;
#13882=DIRECTION ( 'NONE',  ( 0.000000000000000000, 0.000000000000000000, 1.000000000000000000 ) ) ;
#13883=DIRECTION ( 'NONE',  ( 0.000000000000000000, 0.000000000000000000, -1.000000000000000000 ) ) ;
#13885=DIRECTION ( 'NONE',  ( 0.000000000000000000, 1.000000000000000000, 0.000000000000000000 ) ) ;
#13886=DIRECTION ( 'NONE',  ( 0.000000000000000000, -0.000000000000000000, 1.000000000000000000 ) ) ;
#13888=EDGE_CURVE ( 'NONE', #95786, #63967, #72990, .T. ) ;
#13889=VERTEX_POINT ( 'NONE', #126676 ) ;
#13890=DIRECTION ( 'NONE',  ( 0.000000000000000000, 0.000000000000000000, 1.000000000000000000 ) ) ;
#13891=ORIENTED_EDGE ( 'NONE', *, *, #15919, .F. ) ;
#13892=AXIS2_PLACEMENT_3D ( 'NONE', #114495, #45134, #85033 ) ;
#13893=ORIENTED_EDGE ( 'NONE', *, *, #62126, .T. ) ;
#13894=ORIENTED_EDGE ( 'NONE', *, *, #99826, .F. ) ;
#13895=VECTOR ( 'NONE', #94271, 1000.000000000000000 ) ;
#13896=FACE_OUTER_BOUND ( 'NONE', #126561, .T. ) ;
#13897=VERTEX_POINT ( 'NONE', #16689 ) ;
#13898=ORIENTED_EDGE ( 'NONE', *, *, #95079, .F. ) ;
#13899=ORIENTED_EDGE ( 'NONE', *, *, #4781, .F. ) ;
#13900=DIRECTION ( 'NONE',  ( 0.000000000000000000, 0.000000000000000000, 1.000000000000000000 ) ) ;
#13901=CIRCLE ( 'NONE', #59910, 0.06509327318403745899 ) ;
#13902=AXIS2_PLACEMENT_3D ( 'NONE', #100308, #69540, #45572 ) ;
#13903=DIRECTION ( 'NONE',  ( 0.000000000000000000, 0.000000000000000000, 1.000000000000000000 ) ) ;
#13904=DIRECTION ( 'NONE',  ( 0.000000000000000000, 1.000000000000000000, 0.000000000000000000 ) ) ;
#13905=PLANE ( 'NONE',  #31690 ) ;
#13906=LINE ( 'NONE', #85237, #38802 ) ;
#13907=DIRECTION ( 'NONE',  ( 0.000000000000000000, 1.000000000000000000, 0.000000000000000000 ) ) ;
#13908=CARTESIAN_POINT ( 'NONE',  ( 7.899999999999923084, 2.500000000000000000, 0.6928203230275494784 ) ) ;
#13909=CIRCLE ( 'NONE', #126799, 0.09999999999999982514 ) ;
#13910=AXIS2_PLACEMENT_3D ( 'NONE', #780, #41379, #62303 ) ;
#13911=ORIENTED_EDGE ( 'NONE', *, *, #119077, .T. ) ;
#13912=FACE_OUTER_BOUND ( 'NONE', #15011, .T. ) ;
#13913=AXIS2_PLACEMENT_3D ( 'NONE', #64128, #93593, #1980 ) ;
#13914=EDGE_CURVE ( 'NONE', #95931, #129515, #118403, .T. ) ;
#13915=ORIENTED_EDGE ( 'NONE', *, *, #52068, .T. ) ;
#13917=ORIENTED_EDGE ( 'NONE', *, *, #112345, .F. ) ;
#13918=EDGE_LOOP ( 'NONE', ( #98523, #55265 ) ) ;
#13919=EDGE_CURVE ( 'NONE', #14887, #35541, #64116, .T. ) ;
#13920=DIRECTION ( 'NONE',  ( -0.000000000000000000, 1.000000000000000000, -0.000000000000000000 ) ) ;
#13921=DIRECTION ( 'NONE',  ( -4.274815082592931898E-19, -0.9999939076577903929, -0.003490651415223739937 ) ) ;
#13922=DIRECTION ( 'NONE',  ( 0.000000000000000000, 0.000000000000000000, -1.000000000000000000 ) ) ;
#13923=ORIENTED_EDGE ( 'NONE', *, *, #126370, .F. ) ;
#13924=ADVANCED_FACE ( 'NONE', ( #74347 ), #45251, .T. ) ;
#13925=EDGE_CURVE ( 'NONE', #48111, #26681, #86741, .T. ) ;
#13926=VERTEX_POINT ( 'NONE', #76931 ) ;
#13927=CARTESIAN_POINT ( 'NONE',  ( 3.949999999999938893, 12.50000000000000000, 6.083687093685482772 ) ) ;
#13928=CARTESIAN_POINT ( 'NONE',  ( 8.949999999999917577, 12.50000000000000000, -2.511473670974877948 ) ) ;
#13929=EDGE_CURVE ( 'NONE', #104068, #11740, #91224, .T. ) ;
#13930=DIRECTION ( 'NONE',  ( -0.000000000000000000, 1.000000000000000000, -0.000000000000000000 ) ) ;
#13931=EDGE_CURVE ( 'NONE', #11186, #37345, #4288, .T. ) ;
#13932=CONICAL_SURFACE ( 'NONE', #47402, 0.09999999999999982514, 0.003490658503988666988 ) ;
#13933=EDGE_CURVE ( 'NONE', #128871, #98765, #116836, .T. ) ;
#13934=DIRECTION ( 'NONE',  ( -0.000000000000000000, 1.000000000000000000, -0.000000000000000000 ) ) ;
#13935=CARTESIAN_POINT ( 'NONE',  ( -0.4000000000000392131, 2.500000000000000000, -5.122947341949753763 ) ) ;
#13936=ORIENTED_EDGE ( 'NONE', *, *, #113826, .T. ) ;
#13937=B_SPLINE_CURVE_WITH_KNOTS ( 'NONE', 3,
 ( #20442, #100299, #10594, #99653, #81300, #30281, #39467, #121860, #121213, #31555, #79374, #69531, #40751, #50532, #791, #71462 ),
 .UNSPECIFIED., .F., .F.,
 ( 4, 2, 2, 2, 2, 2, 2, 4 ),
 ( 0.000000000000000000, 0.0008828639377709713437, 0.001765727875541942687, 0.003531455751083888411, 0.005297183626625834134, 0.007062911502167780291, 0.01059436725325167694, 0.01412582300433557272 ),
 .UNSPECIFIED. ) ;
#13938=EDGE_CURVE ( 'NONE', #82940, #65438, #70384, .T. ) ;
#13939=EDGE_LOOP ( 'NONE', ( #35323, #31126, #128553, #105815 ) ) ;
#13940=CIRCLE ( 'NONE', #49483, 0.06509327318403745899 ) ;
#13941=EDGE_CURVE ( 'NONE', #121566, #84561, #107942, .T. ) ;
#13942=DIRECTION ( 'NONE',  ( -0.000000000000000000, -1.000000000000000000, -0.000000000000000000 ) ) ;
#13943=DIRECTION ( 'NONE',  ( -0.000000000000000000, -1.000000000000000000, -0.000000000000000000 ) ) ;
#13944=EDGE_CURVE ( 'NONE', #10631, #41518, #32752, .T. ) ;
#13945=AXIS2_PLACEMENT_3D ( 'NONE', #127776, #118597, #38117 ) ;
#13947=LINE ( 'NONE', #114731, #36464 ) ;
#13948=VECTOR ( 'NONE', #51096, 1000.000000000000000 ) ;
#13949=FACE_OUTER_BOUND ( 'NONE', #60071, .T. ) ;
#13950=FACE_OUTER_BOUND ( 'NONE', #87132, .T. ) ;
#13951=DIRECTION ( 'NONE',  ( -0.000000000000000000, -1.000000000000000000, -0.000000000000000000 ) ) ;
#13952=EDGE_LOOP ( 'NONE', ( #89486, #20805, #69898, #17945 ) ) ;
#13953=CIRCLE ( 'NONE', #112171, 0.06509327318403745899 ) ;
#13954=CARTESIAN_POINT ( 'NONE',  ( -13.34999999999999076, 12.50000000000000000, -2.165063509461099489 ) ) ;
#13955=CIRCLE ( 'NONE', #85067, 0.06509327318403745899 ) ;
#13956=CIRCLE ( 'NONE', #24433, 0.09999999999999982514 ) ;
#13957=DIRECTION ( 'NONE',  ( 0.000000000000000000, -0.9999939076577903929, 0.003490651415223739937 ) ) ;
#13958=CARTESIAN_POINT ( 'NONE',  ( 0.8499999999999553468, 2.500000000000000000, -2.757883832488654097 ) ) ;
#13960=CARTESIAN_POINT ( 'NONE',  ( 9.799999999999913669, 12.50000000000000000, 4.676537180435972552 ) ) ;
#13961=EDGE_LOOP ( 'NONE', ( #112653, #80659 ) ) ;
#13962=CARTESIAN_POINT ( 'NONE',  ( -1.900000000000034106, 2.500000000000000000, 0.3464101615137735735 ) ) ;
#13963=ORIENTED_EDGE ( 'NONE', *, *, #94959, .T. ) ;
#13964=DIRECTION ( 'NONE',  ( 0.000000000000000000, 0.000000000000000000, 1.000000000000000000 ) ) ;
#13965=DIRECTION ( 'NONE',  ( 0.000000000000000000, 0.000000000000000000, 1.000000000000000000 ) ) ;
#13966=AXIS2_PLACEMENT_3D ( 'NONE', #92777, #73754, #13549 ) ;
#13967=CARTESIAN_POINT ( 'NONE',  ( 8.349999999999919709, 2.500000000000000000, -2.857883832488653741 ) ) ;
#13968=VERTEX_POINT ( 'NONE', #108943 ) ;
#13969=DIRECTION ( 'NONE',  ( 0.000000000000000000, -0.000000000000000000, 1.000000000000000000 ) ) ;
#13970=CARTESIAN_POINT ( 'NONE',  ( -8.950000000000009948, 2.500000000000000000, 2.411473670974873862 ) ) ;
#13971=EDGE_CURVE ( 'NONE', #6869, #86595, #37660, .T. ) ;
#13973=EDGE_CURVE ( 'NONE', #9476, #13889, #27818, .T. ) ;
#13974=AXIS2_PLACEMENT_3D ( 'NONE', #18872, #8402, #36613 ) ;
#13975=ORIENTED_EDGE ( 'NONE', *, *, #103601, .T. ) ;
#13976=VECTOR ( 'NONE', #99453, 1000.000000000000000 ) ;
#13977=EDGE_CURVE ( 'NONE', #20697, #13290, #20215, .T. ) ;
#13978=EDGE_LOOP ( 'NONE', ( #83134, #43120 ) ) ;
#13979=FACE_OUTER_BOUND ( 'NONE', #91749, .T. ) ;
#13980=DIRECTION ( 'NONE',  ( 0.000000000000000000, -0.000000000000000000, 1.000000000000000000 ) ) ;
#13981=DIRECTION ( 'NONE',  ( -0.000000000000000000, 1.000000000000000000, -0.000000000000000000 ) ) ;
#13982=ORIENTED_EDGE ( 'NONE', *, *, #10418, .F. ) ;
#13983=CARTESIAN_POINT ( 'NONE',  ( 2.099999999999948574, 2.500000000000000000, 3.637306695894644726 ) ) ;
#13985=VERTEX_POINT ( 'NONE', #120085 ) ;
#13986=EDGE_CURVE ( 'NONE', #27533, #41344, #99631, .T. ) ;
#13987=VECTOR ( 'NONE', #42467, 1000.000000000000000 ) ;
#13988=DIRECTION ( 'NONE',  ( -0.000000000000000000, -1.000000000000000000, -0.000000000000000000 ) ) ;
#13989=DIRECTION ( 'NONE',  ( 0.000000000000000000, 0.000000000000000000, 1.000000000000000000 ) ) ;
#13990=FACE_OUTER_BOUND ( 'NONE', #14692, .T. ) ;
#13991=DIRECTION ( 'NONE',  ( 0.000000000000000000, 1.000000000000000000, 0.000000000000000000 ) ) ;
#13992=DIRECTION ( 'NONE',  ( 0.000000000000000000, 0.000000000000000000, 1.000000000000000000 ) ) ;
#13993=CARTESIAN_POINT ( 'NONE',  ( -4.400000000000028777, 12.50000000000000000, -3.918623584224389056 ) ) ;
#13994=CARTESIAN_POINT ( 'NONE',  ( -10.60000000000000142, 12.50000000000000000, 0.3464101615137736845 ) ) ;
#13995=AXIS2_PLACEMENT_3D ( 'NONE', #96897, #38656, #78575 ) ;
#13996=CONICAL_SURFACE ( 'NONE', #60014, 0.1000000000000000472, 0.003490658503988666988 ) ;
#13997=ORIENTED_EDGE ( 'NONE', *, *, #86402, .F. ) ;
#13998=ORIENTED_EDGE ( 'NONE', *, *, #9634, .T. ) ;
#13999=ORIENTED_EDGE ( 'NONE', *, *, #122429, .F. ) ;
#14000=ORIENTED_EDGE ( 'NONE', *, *, #108363, .F. ) ;
#14001=FACE_OUTER_BOUND ( 'NONE', #41097, .T. ) ;
#14002=FACE_OUTER_BOUND ( 'NONE', #6717, .T. ) ;
#14003=DIRECTION ( 'NONE',  ( -4.274815082592931898E-19, -0.9999939076577903929, -0.003490651415223739937 ) ) ;
#14004=EDGE_LOOP ( 'NONE', ( #86123, #45825, #7526, #66310 ) ) ;
#14005=FACE_BOUND ( 'NONE', #123227, .T. ) ;
#14006=ADVANCED_FACE ( 'NONE', ( #89330 ), #112156, .T. ) ;
#14007=DIRECTION ( 'NONE',  ( 0.000000000000000000, 0.000000000000000000, 1.000000000000000000 ) ) ;
#14008=CARTESIAN_POINT ( 'NONE',  ( 7.699999999999925571, 12.50000000000000000, -4.676537180435978769 ) ) ;
#14009=CARTESIAN_POINT ( 'NONE',  ( -10.60000000000000142, 2.500000000000000000, 0.3464101615137736845 ) ) ;
#14011=CARTESIAN_POINT ( 'NONE',  ( -2.100000000000033396, 12.50000000000000000, -3.702399969078687292 ) ) ;
#14012=DIRECTION ( 'NONE',  ( -0.000000000000000000, 1.000000000000000000, -0.000000000000000000 ) ) ;
#14013=FACE_OUTER_BOUND ( 'NONE', #61402, .T. ) ;
#14014=DIRECTION ( 'NONE',  ( 0.000000000000000000, 0.000000000000000000, 1.000000000000000000 ) ) ;
#14016=AXIS2_PLACEMENT_3D ( 'NONE', #4509, #85676, #84392 ) ;
#14017=CIRCLE ( 'NONE', #64199, 0.06509327318403745899 ) ;
#14018=CARTESIAN_POINT ( 'NONE',  ( 2.099999999999948574, 2.500000000000000000, 4.330127018922196314 ) ) ;
#14020=EDGE_LOOP ( 'NONE', ( #109836, #101801, #24691, #90109 ) ) ;
#14021=AXIS2_PLACEMENT_3D ( 'NONE', #53914, #29601, #127803 ) ;
#14022=ORIENTED_EDGE ( 'NONE', *, *, #43676, .F. ) ;
#14023=EDGE_CURVE ( 'NONE', #23927, #67054, #41166, .T. ) ;
#14024=ORIENTED_EDGE ( 'NONE', *, *, #124315, .F. ) ;
#14026=ORIENTED_EDGE ( 'NONE', *, *, #35455, .F. ) ;
#14027=FACE_OUTER_BOUND ( 'NONE', #10077, .T. ) ;
#14028=VERTEX_POINT ( 'NONE', #20590 ) ;
#14029=CONICAL_SURFACE ( 'NONE', #68412, 0.09999999999999982514, 0.003490658503988666988 ) ;
#14030=ORIENTED_EDGE ( 'NONE', *, *, #72648, .T. ) ;
#14031=CARTESIAN_POINT ( 'NONE',  ( 12.65326442612073166, -2.500000000000508038, 8.428886917615358243 ) ) ;
#14032=CARTESIAN_POINT ( 'NONE',  ( 0.8499999999999550138, 12.50000000000000000, -5.802370205355749988 ) ) ;
#14033=DIRECTION ( 'NONE',  ( -4.274815082592931898E-19, -0.9999939076577903929, -0.003490651415223739937 ) ) ;
#14034=EDGE_CURVE ( 'NONE', #122281, #111372, #68221, .T. ) ;
#14035=ORIENTED_EDGE ( 'NONE', *, *, #128982, .T. ) ;
#14036=DIRECTION ( 'NONE',  ( 0.000000000000000000, -0.9999939076577903929, 0.003490651415223739937 ) ) ;
#14037=EDGE_LOOP ( 'NONE', ( #78181, #9378, #69485, #119446 ) ) ;
#14038=VECTOR ( 'NONE', #125311, 1000.000000000000000 ) ;
#14039=CIRCLE ( 'NONE', #51721, 0.06509327318403745899 ) ;
#14040=ORIENTED_EDGE ( 'NONE', *, *, #459, .T. ) ;
#14041=FACE_OUTER_BOUND ( 'NONE', #126694, .T. ) ;
#14042=ORIENTED_EDGE ( 'NONE', *, *, #75702, .F. ) ;
#14044=ORIENTED_EDGE ( 'NONE', *, *, #59194, .T. ) ;
#14046=CARTESIAN_POINT ( 'NONE',  ( -6.700000000000019718, 2.500000000000000000, -2.385244779468109755E-15 ) ) ;
#14047=DIRECTION ( 'NONE',  ( -0.000000000000000000, 1.000000000000000000, -0.000000000000000000 ) ) ;
#14048=DIRECTION ( 'NONE',  ( 0.000000000000000000, 0.000000000000000000, 1.000000000000000000 ) ) ;
#14049=CARTESIAN_POINT ( 'NONE',  ( 1.449999999999949551, 2.500000000000000000, 6.741600689897071952 ) ) ;
#14050=LINE ( 'NONE', #15985, #127640 ) ;
#14051=AXIS2_PLACEMENT_3D ( 'NONE', #99222, #89396, #29206 ) ;
#14052=ORIENTED_EDGE ( 'NONE', *, *, #111186, .T. ) ;
#14053=LINE ( 'NONE', #54006, #107547 ) ;
#14054=ORIENTED_EDGE ( 'NONE', *, *, #11463, .T. ) ;
#14055=CARTESIAN_POINT ( 'NONE',  ( 87.50000000000001421, 4.424430252271040587, -6.079088403633664761 ) ) ;
#14056=ADVANCED_FACE ( 'NONE', ( #49417 ), #24415, .T. ) ;
#14057=VERTEX_POINT ( 'NONE', #39611 ) ;
#14058=CARTESIAN_POINT ( 'NONE',  ( 4.149999999999938183, 2.500000000000000000, 2.065063509461097624 ) ) ;
#14059=CARTESIAN_POINT ( 'NONE',  ( 0.000000000000000000, 1.500000000000000000, -8.999999999999998224 ) ) ;
#14060=CARTESIAN_POINT ( 'NONE',  ( 8.299999999999922551, 12.50000000000000000, 4.330127018922196314 ) ) ;
#14061=DIRECTION ( 'NONE',  ( 0.000000000000000000, 1.000000000000000000, 0.000000000000000000 ) ) ;
#14062=ORIENTED_EDGE ( 'NONE', *, *, #52955, .F. ) ;
#14063=EDGE_CURVE ( 'NONE', #114185, #115197, #82912, .T. ) ;
#14064=( NAMED_UNIT ( * ) SI_UNIT ( $, .STERADIAN. ) SOLID_ANGLE_UNIT ( ) );
#14065=AXIS2_PLACEMENT_3D ( 'NONE', #74435, #35166, #94703 ) ;
#14066=AXIS2_PLACEMENT_3D ( 'NONE', #81427, #33610, #72258 ) ;
#14067=CARTESIAN_POINT ( 'NONE',  ( -13.54999999999999005, 12.50000000000000000, 2.446380397790839822 ) ) ;
#14068=EDGE_LOOP ( 'NONE', ( #98199, #129505, #22050, #57791 ) ) ;
#14069=ORIENTED_EDGE ( 'NONE', *, *, #6834, .F. ) ;
#14070=EDGE_CURVE ( 'NONE', #51458, #78977, #97845, .T. ) ;
#14071=ADVANCED_FACE ( 'NONE', ( #109620 ), #101691, .T. ) ;
#14072=EDGE_LOOP ( 'NONE', ( #72679, #31100 ) ) ;
#14073=FACE_OUTER_BOUND ( 'NONE', #65009, .T. ) ;
#14074=FACE_OUTER_BOUND ( 'NONE', #96061, .T. ) ;
#14075=ADVANCED_FACE ( 'NONE', ( #10126 ), #87092, .T. ) ;
#14077=EDGE_CURVE ( 'NONE', #54383, #105257, #28479, .T. ) ;
#14078=LINE ( 'NONE', #122134, #1016 ) ;
#14079=CONICAL_SURFACE ( 'NONE', #26617, 0.09999999999999982514, 0.003490658503988666988 ) ;
#14080=VECTOR ( 'NONE', #116324, 1000.000000000000000 ) ;
#14081=CIRCLE ( 'NONE', #97717, 0.09999999999999999167 ) ;
#14082=LINE ( 'NONE', #63203, #105398 ) ;
#14083=PLANE ( 'NONE',  #94456 ) ;
#14084=EDGE_CURVE ( 'NONE', #72875, #43830, #18138, .T. ) ;
#14085=ADVANCED_FACE ( 'NONE', ( #118136 ), #110089, .T. ) ;
#14086=EDGE_CURVE ( 'NONE', #121533, #111424, #110253, .T. ) ;
#14087=CIRCLE ( 'NONE', #1574, 0.1000000000000002554 ) ;
#14088=CIRCLE ( 'NONE', #59830, 0.1000000000000002554 ) ;
#14089=ORIENTED_EDGE ( 'NONE', *, *, #32620, .T. ) ;
#14090=EDGE_CURVE ( 'NONE', #32421, #21428, #128903, .T. ) ;
#14091=PLANE ( 'NONE',  #115417 ) ;
#14092=AXIS2_PLACEMENT_3D ( 'NONE', #56512, #29007, #68911 ) ;
#14093=EDGE_CURVE ( 'NONE', #90527, #113481, #126816, .T. ) ;
#14094=ORIENTED_EDGE ( 'NONE', *, *, #110465, .F. ) ;
#14095=FACE_OUTER_BOUND ( 'NONE', #46471, .T. ) ;
#14096=FACE_OUTER_BOUND ( 'NONE', #87873, .T. ) ;
#14097=DIRECTION ( 'NONE',  ( 0.000000000000000000, 1.000000000000000000, 0.000000000000000000 ) ) ;
#14098=CARTESIAN_POINT ( 'NONE',  ( -4.600000000000028066, 2.500000000000000000, -5.022947341949754119 ) ) ;
#14099=EDGE_CURVE ( 'NONE', #88292, #121575, #47409, .T. ) ;
#14100=EDGE_LOOP ( 'NONE', ( #78539, #37288 ) ) ;
#14101=AXIS2_PLACEMENT_3D ( 'NONE', #72960, #110927, #70375 ) ;
#14102=FACE_OUTER_BOUND ( 'NONE', #47291, .T. ) ;
#14103=DIRECTION ( 'NONE',  ( 0.000000000000000000, 0.000000000000000000, -1.000000000000000000 ) ) ;
#14104=ORIENTED_EDGE ( 'NONE', *, *, #57355, .T. ) ;
#14105=AXIS2_PLACEMENT_3D ( 'NONE', #38697, #126408, #6590 ) ;
#14106=AXIS2_PLACEMENT_3D ( 'NONE', #35939, #105967, #14348 ) ;
#14107=VERTEX_POINT ( 'NONE', #21894 ) ;
#14108=FACE_OUTER_BOUND ( 'NONE', #48034, .T. ) ;
#14109=AXIS2_PLACEMENT_3D ( 'NONE', #61797, #72262, #91889 ) ;
#14110=ORIENTED_EDGE ( 'NONE', *, *, #61238, .F. ) ;
#14111=ORIENTED_EDGE ( 'NONE', *, *, #7424, .F. ) ;
#14112=DIRECTION ( 'NONE',  ( 0.000000000000000000, -0.000000000000000000, 1.000000000000000000 ) ) ;
#14114=ORIENTED_EDGE ( 'NONE', *, *, #105446, .T. ) ;
#14115=DIRECTION ( 'NONE',  ( -4.274815082592931898E-19, -0.9999939076577903929, -0.003490651415223739937 ) ) ;
#14116=CARTESIAN_POINT ( 'NONE',  ( -11.04999999999999893, 2.500000000000000000, 6.248780366869520542 ) ) ;
#14117=AXIS2_PLACEMENT_3D ( 'NONE', #13382, #62511, #92598 ) ;
#14118=CARTESIAN_POINT ( 'NONE',  ( -10.84999999999999964, 2.500000000000000000, 7.088010851410848190 ) ) ;
#14119=VERTEX_POINT ( 'NONE', #122016 ) ;
#14120=CIRCLE ( 'NONE', #35004, 0.09999999999999999167 ) ;
#14121=AXIS2_PLACEMENT_3D ( 'NONE', #102669, #13641, #102041 ) ;
#14122=DIRECTION ( 'NONE',  ( 0.000000000000000000, -0.9999939076577903929, 0.003490651415223739937 ) ) ;
#14123=CARTESIAN_POINT ( 'NONE',  ( 12.94999999999989981, 2.500000000000000000, -2.265063509461101798 ) ) ;
#14124=VERTEX_POINT ( 'NONE', #72280 ) ;
#14125=CARTESIAN_POINT ( 'NONE',  ( 5.449999999999934452, 12.50000000000000000, 2.230156782645134950 ) ) ;
#14126=AXIS2_PLACEMENT_3D ( 'NONE', #24051, #93431, #54152 ) ;
#14127=DIRECTION ( 'NONE',  ( -0.000000000000000000, 1.000000000000000000, -0.000000000000000000 ) ) ;
#14128=ORIENTED_EDGE ( 'NONE', *, *, #111024, .T. ) ;
#14129=EDGE_CURVE ( 'NONE', #75768, #128878, #112190, .T. ) ;
#14130=AXIS2_PLACEMENT_3D ( 'NONE', #49357, #89254, #39547 ) ;
#14131=AXIS2_PLACEMENT_3D ( 'NONE', #85285, #6067, #75460 ) ;
#14132=EDGE_LOOP ( 'NONE', ( #67047, #88585, #5866, #28705 ) ) ;
#14133=EDGE_CURVE ( 'NONE', #51338, #81852, #26476, .T. ) ;
#14134=EDGE_LOOP ( 'NONE', ( #87226, #31430 ) ) ;
#14135=ORIENTED_EDGE ( 'NONE', *, *, #17592, .T. ) ;
#14136=DIRECTION ( 'NONE',  ( 0.000000000000000000, 0.000000000000000000, 1.000000000000000000 ) ) ;
#14137=DIRECTION ( 'NONE',  ( 0.000000000000000000, 0.000000000000000000, -1.000000000000000000 ) ) ;
#14138=PLANE ( 'NONE',  #8646 ) ;
#14139=FACE_BOUND ( 'NONE', #75103, .T. ) ;
#14140=VERTEX_POINT ( 'NONE', #103002 ) ;
#14142=DIRECTION ( 'NONE',  ( -0.000000000000000000, 1.000000000000000000, -0.000000000000000000 ) ) ;
#14143=CARTESIAN_POINT ( 'NONE',  ( 8.749999999999953815, 2.500000000000000000, 6.495190528383297135 ) ) ;
#14144=EDGE_CURVE ( 'NONE', #11222, #107586, #120556, .T. ) ;
#14145=CARTESIAN_POINT ( 'NONE',  ( 0.8499999999999557909, 2.500000000000000000, -6.495190528383302464 ) ) ;
#14146=CARTESIAN_POINT ( 'NONE',  ( -4.350000000000023626, 12.50000000000000000, 1.753560074763284016 ) ) ;
#14147=AXIS2_PLACEMENT_3D ( 'NONE', #107878, #28689, #78448 ) ;
#14148=CARTESIAN_POINT ( 'NONE',  ( -1.450000000000036371, 2.500000000000000000, 2.511473670974873507 ) ) ;
#14149=CARTESIAN_POINT ( 'NONE',  ( 10.84999999999990905, 2.500000000000000000, -5.702370205355749455 ) ) ;
#14150=ORIENTED_EDGE ( 'NONE', *, *, #113564, .F. ) ;
#14151=ORIENTED_EDGE ( 'NONE', *, *, #121385, .T. ) ;
#14152=ORIENTED_EDGE ( 'NONE', *, *, #127164, .T. ) ;
#14154=ORIENTED_EDGE ( 'NONE', *, *, #104839, .F. ) ;
#14155=DIRECTION ( 'NONE',  ( 0.000000000000000000, -0.9999939076577903929, 0.003490651415223739937 ) ) ;
#14156=CARTESIAN_POINT ( 'NONE',  ( 8.749999999999918288, 12.50000000000000000, 7.122917578226811486 ) ) ;
#14157=ORIENTED_EDGE ( 'NONE', *, *, #18720, .F. ) ;
#14158=FACE_BOUND ( 'NONE', #93206, .T. ) ;
#14159=FACE_OUTER_BOUND ( 'NONE', #33240, .T. ) ;
#14160=CIRCLE ( 'NONE', #33078, 0.1000000000000000472 ) ;
#14161=AXIS2_PLACEMENT_3D ( 'NONE', #40053, #99623, #60352 ) ;
#14162=ORIENTED_EDGE ( 'NONE', *, *, #6247, .F. ) ;
#14163=CARTESIAN_POINT ( 'NONE',  ( 12.69999999999989981, 2.500000000000000000, -0.4464101615137783252 ) ) ;
#14164=CARTESIAN_POINT ( 'NONE',  ( 4.799999999999939426, 12.50000000000000000, -4.676537180435977881 ) ) ;
#14165=DIRECTION ( 'NONE',  ( -0.000000000000000000, -1.000000000000000000, -0.000000000000000000 ) ) ;
#14166=EDGE_LOOP ( 'NONE', ( #86658, #20625, #26215, #43059 ) ) ;
#14167=CARTESIAN_POINT ( 'NONE',  ( 15.83209681635537258, -2.500000000000000000, 5.404881881984331393 ) ) ;
#14168=AXIS2_PLACEMENT_3D ( 'NONE', #88161, #78388, #118293 ) ;
#14169=EDGE_CURVE ( 'NONE', #74255, #78385, #74586, .T. ) ;
#14170=ORIENTED_EDGE ( 'NONE', *, *, #91259, .T. ) ;
#14171=CONICAL_SURFACE ( 'NONE', #122860, 0.1000000000000002554, 0.003490658503988666988 ) ;
#14172=CONICAL_SURFACE ( 'NONE', #120799, 0.1000000000000002554, 0.003490658503988666988 ) ;
#14173=VERTEX_POINT ( 'NONE', #12679 ) ;
#14174=VERTEX_POINT ( 'NONE', #11405 ) ;
#14175=DIRECTION ( 'NONE',  ( -0.000000000000000000, -1.000000000000000000, -0.000000000000000000 ) ) ;
#14176=FACE_OUTER_BOUND ( 'NONE', #10379, .T. ) ;
#14177=DIRECTION ( 'NONE',  ( 0.000000000000000000, -0.9999939076577903929, 0.003490651415223739937 ) ) ;
#14178=ORIENTED_EDGE ( 'NONE', *, *, #108057, .T. ) ;
#14179=DIRECTION ( 'NONE',  ( 0.000000000000000000, 1.000000000000000000, 0.000000000000000000 ) ) ;
#14180=CIRCLE ( 'NONE', #1667, 0.09999999999999999167 ) ;
#14181=CARTESIAN_POINT ( 'NONE',  ( 11.69999999999990870, 2.500000000000000000, 4.230127018922196669 ) ) ;
#14182=DIRECTION ( 'NONE',  ( 0.000000000000000000, 0.000000000000000000, -1.000000000000000000 ) ) ;
#14184=ORIENTED_EDGE ( 'NONE', *, *, #88580, .F. ) ;
#14185=EDGE_CURVE ( 'NONE', #25038, #5720, #28623, .T. ) ;
#14186=FACE_OUTER_BOUND ( 'NONE', #24380, .T. ) ;
#14187=EDGE_CURVE ( 'NONE', #83267, #72199, #53745, .T. ) ;
#14188=ORIENTED_EDGE ( 'NONE', *, *, #24004, .T. ) ;
#14189=DIRECTION ( 'NONE',  ( 0.000000000000000000, 0.000000000000000000, 1.000000000000000000 ) ) ;
#14190=CIRCLE ( 'NONE', #47671, 0.06509327318403745899 ) ;
#14191=EDGE_LOOP ( 'NONE', ( #78000, #123029 ) ) ;
#14192=ORIENTED_EDGE ( 'NONE', *, *, #22092, .F. ) ;
#14193=CARTESIAN_POINT ( 'NONE',  ( -0.2000000000000399791, 2.500000000000000000, -4.776537180435977525 ) ) ;
#14194=AXIS2_PLACEMENT_3D ( 'NONE', #31613, #11320, #122572 ) ;
#14195=CARTESIAN_POINT ( 'NONE',  ( 1.649999999999950617, 2.500000000000000000, 2.165063509461097713 ) ) ;
#14196=FACE_OUTER_BOUND ( 'NONE', #10802, .T. ) ;
#14197=DIRECTION ( 'NONE',  ( 0.000000000000000000, 1.000000000000000000, 0.000000000000000000 ) ) ;
#14198=ADVANCED_FACE ( 'NONE', ( #10734 ), #128995, .T. ) ;
#14199=CARTESIAN_POINT ( 'NONE',  ( -0.6000000000000323963, 2.500000000000000000, -0.4464101615137759382 ) ) ;
#14200=CONICAL_SURFACE ( 'NONE', #62352, 0.09999999999999999167, 0.003490658503988666988 ) ;
#14201=ORIENTED_EDGE ( 'NONE', *, *, #85223, .F. ) ;
#14202=AXIS2_PLACEMENT_3D ( 'NONE', #13725, #63492, #112597 ) ;
#14203=EDGE_LOOP ( 'NONE', ( #86550, #30054, #8122, #52219 ) ) ;
#14205=CIRCLE ( 'NONE', #45533, 0.1000000000000002554 ) ;
#14207=FACE_OUTER_BOUND ( 'NONE', #93588, .T. ) ;
#14208=ORIENTED_EDGE ( 'NONE', *, *, #38903, .T. ) ;
#14209=EDGE_LOOP ( 'NONE', ( #21954, #94314, #83194, #109520 ) ) ;
#14210=DIRECTION ( 'NONE',  ( 0.000000000000000000, 1.000000000000000000, 0.000000000000000000 ) ) ;
#14211=CIRCLE ( 'NONE', #24700, 0.06509327318403745899 ) ;
#14212=AXIS2_PLACEMENT_3D ( 'NONE', #7422, #109505, #59791 ) ;
#14213=VERTEX_POINT ( 'NONE', #92541 ) ;
#14216=EDGE_LOOP ( 'NONE', ( #83478, #101961 ) ) ;
#14217=CARTESIAN_POINT ( 'NONE',  ( -12.69999999999999218, 2.500000000000000000, 4.676537180435972552 ) ) ;
#14218=CARTESIAN_POINT ( 'NONE',  ( -3.469446951953614189E-14, 12.50000000000000000, -0.6928203230275519209 ) ) ;
#14219=DIRECTION ( 'NONE',  ( -0.000000000000000000, 1.000000000000000000, -0.000000000000000000 ) ) ;
#14220=AXIS2_PLACEMENT_3D ( 'NONE', #42023, #64234, #21743 ) ;
#14221=CARTESIAN_POINT ( 'NONE',  ( -0.6000000000000323963, 12.50000000000000000, -0.3464101615137759604 ) ) ;
#14222=ORIENTED_EDGE ( 'NONE', *, *, #5113, .T. ) ;
#14223=EDGE_CURVE ( 'NONE', #21908, #111830, #120652, .T. ) ;
#14224=FACE_OUTER_BOUND ( 'NONE', #28477, .T. ) ;
#14225=CONICAL_SURFACE ( 'NONE', #26763, 0.09999999999999982514, 0.003490658503988666988 ) ;
#14226=VECTOR ( 'NONE', #112667, 1000.000000000000000 ) ;
#14227=CARTESIAN_POINT ( 'NONE',  ( 26.76314062975269081, -1.072173157150710043, 4.440523076943300396 ) ) ;
#14230=ORIENTED_EDGE ( 'NONE', *, *, #127488, .T. ) ;
#14231=EDGE_CURVE ( 'NONE', #47341, #41439, #80807, .T. ) ;
#14233=DIRECTION ( 'NONE',  ( 0.000000000000000000, 0.000000000000000000, 1.000000000000000000 ) ) ;
#14234=FACE_OUTER_BOUND ( 'NONE', #106693, .T. ) ;
#14235=ADVANCED_FACE ( 'NONE', ( #120719 ), #63086, .T. ) ;
#14236=DIRECTION ( 'NONE',  ( 0.000000000000000000, 0.000000000000000000, 1.000000000000000000 ) ) ;
#14237=FACE_OUTER_BOUND ( 'NONE', #10479, .T. ) ;
#14238=CARTESIAN_POINT ( 'NONE',  ( -0.6000000000000388356, 2.500000000000000000, 4.576537180435972019 ) ) ;
#14239=DIRECTION ( 'NONE',  ( 0.000000000000000000, 1.000000000000000000, 0.000000000000000000 ) ) ;
#14240=DIRECTION ( 'NONE',  ( 0.000000000000000000, 0.000000000000000000, 1.000000000000000000 ) ) ;
#14241=CARTESIAN_POINT ( 'NONE',  ( 4.799999999999939426, 2.500000000000000000, -4.776537180435977525 ) ) ;
#14242=DIRECTION ( 'NONE',  ( 0.000000000000000000, -0.9999939076577903929, 0.003490651415223739937 ) ) ;
#14243=EDGE_CURVE ( 'NONE', #108419, #84285, #31702, .T. ) ;
#14244=ADVANCED_FACE ( 'NONE', ( #51992 ), #64202, .T. ) ;
#14245=EDGE_CURVE ( 'NONE', #1262, #111853, #49558, .T. ) ;
#14246=LINE ( 'NONE', #83020, #12476 ) ;
#14247=VERTEX_POINT ( 'NONE', #123296 ) ;
#14248=ORIENTED_EDGE ( 'NONE', *, *, #53884, .F. ) ;
#14249=EDGE_CURVE ( 'NONE', #2581, #107840, #45359, .T. ) ;
#14250=EDGE_LOOP ( 'NONE', ( #14464, #27483 ) ) ;
#14251=CIRCLE ( 'NONE', #24732, 0.1000000000000002554 ) ;
#14252=VECTOR ( 'NONE', #115598, 1000.000000000000000 ) ;
#14253=EDGE_LOOP ( 'NONE', ( #3330, #75026 ) ) ;
#14254=EDGE_CURVE ( 'NONE', #85684, #17230, #122707, .T. ) ;
#14255=DIRECTION ( 'NONE',  ( -0.000000000000000000, -1.000000000000000000, -0.000000000000000000 ) ) ;
#14256=CARTESIAN_POINT ( 'NONE',  ( -4.400000000000028777, 2.500000000000000000, -4.776537180435978414 ) ) ;
#14257=ADVANCED_FACE ( 'NONE', ( #106237 ), #34293, .T. ) ;
#14258=ORIENTED_EDGE ( 'NONE', *, *, #51331, .F. ) ;
#14259=CONICAL_SURFACE ( 'NONE', #118825, 0.1000000000000002554, 0.003490658503988666988 ) ;
#14260=CARTESIAN_POINT ( 'NONE',  ( 1.049999999999954525, 2.500000000000000000, -2.511473670974877948 ) ) ;
#14261=AXIS2_PLACEMENT_3D ( 'NONE', #36027, #74657, #15725 ) ;
#14262=CARTESIAN_POINT ( 'NONE',  ( -4.350000000000023626, 12.50000000000000000, 2.446380397790835826 ) ) ;
#14264=EDGE_LOOP ( 'NONE', ( #124137, #24173, #116378, #44428 ) ) ;
#14265=CARTESIAN_POINT ( 'NONE',  ( 13.74999999999989697, 12.50000000000000000, 2.857883832488649301 ) ) ;
#14266=VECTOR ( 'NONE', #46336, 1000.000000000000000 ) ;
#14267=CARTESIAN_POINT ( 'NONE',  ( 2.699999999999944666, 2.500000000000000000, 4.776537180435972196 ) ) ;
#14269=AXIS2_PLACEMENT_3D ( 'NONE', #123708, #91051, #62886 ) ;
#14270=VERTEX_POINT ( 'NONE', #14608 ) ;
#14271=ORIENTED_EDGE ( 'NONE', *, *, #86744, .F. ) ;
#14272=EDGE_LOOP ( 'NONE', ( #28358, #41243, #38757, #52642 ) ) ;
#14273=CARTESIAN_POINT ( 'NONE',  ( -10.40000000000000213, 2.500000000000000000, -4.330127018922197202 ) ) ;
#14274=CARTESIAN_POINT ( 'NONE',  ( 3.099999999999945466, 2.500000000000000000, -4.083716857408426826 ) ) ;
#14275=CARTESIAN_POINT ( 'NONE',  ( 15.19999999999989093, 2.500000000000000000, 0.3464101615137735735 ) ) ;
#14276=LINE ( 'NONE', #54222, #114675 ) ;
#14277=VECTOR ( 'NONE', #30145, 1000.000000000000000 ) ;
#14278=EDGE_LOOP ( 'NONE', ( #22363, #96196, #63227, #31646 ) ) ;
#14279=CARTESIAN_POINT ( 'NONE',  ( 12.29999999999990656, 2.500000000000000000, -4.676537180435977881 ) ) ;
#14280=ORIENTED_EDGE ( 'NONE', *, *, #70683, .F. ) ;
#14281=VECTOR ( 'NONE', #21178, 1000.000000000000000 ) ;
#14282=DIRECTION ( 'NONE',  ( 0.000000000000000000, -0.9999939076577903929, 0.003490651415223739937 ) ) ;
#14283=FACE_OUTER_BOUND ( 'NONE', #29084, .T. ) ;
#14284=CARTESIAN_POINT ( 'NONE',  ( 4.599999999999939249, 2.500000000000000000, -3.637306695894650055 ) ) ;
#14285=CARTESIAN_POINT ( 'NONE',  ( 6.699999999999930012, 2.500000000000000000, -4.430127018922202176 ) ) ;
#14286=ORIENTED_EDGE ( 'NONE', *, *, #127988, .F. ) ;
#14287=CIRCLE ( 'NONE', #112513, 0.1000000000000002554 ) ;
#14288=EDGE_CURVE ( 'NONE', #95225, #88750, #116428, .T. ) ;
#14289=VERTEX_POINT ( 'NONE', #63741 ) ;
#14290=ORIENTED_EDGE ( 'NONE', *, *, #69105, .T. ) ;
#14291=CARTESIAN_POINT ( 'NONE',  ( -1.250000000000036193, 12.50000000000000000, 1.537336459617582918 ) ) ;
#14292=CARTESIAN_POINT ( 'NONE',  ( -6.050000000000020250, 12.50000000000000000, -2.446380397790840266 ) ) ;
#14293=CARTESIAN_POINT ( 'NONE',  ( -4.400000000000028777, 2.500000000000000000, -3.983716857408426293 ) ) ;
#14294=FACE_BOUND ( 'NONE', #108517, .T. ) ;
#14295=DIRECTION ( 'NONE',  ( 0.000000000000000000, 1.000000000000000000, 0.000000000000000000 ) ) ;
#14296=LINE ( 'NONE', #53605, #40249 ) ;
#14297=DIRECTION ( 'NONE',  ( 0.000000000000000000, -0.9999939076577903929, 0.003490651415223739937 ) ) ;
#14298=EDGE_CURVE ( 'NONE', #88991, #102186, #18234, .T. ) ;
#14299=AXIS2_PLACEMENT_3D ( 'NONE', #91080, #1405, #121184 ) ;
#14301=CARTESIAN_POINT ( 'NONE',  ( 3.349999999999944578, 12.50000000000000000, -5.867463478539787225 ) ) ;
#14302=CONICAL_SURFACE ( 'NONE', #87464, 0.09999999999999982514, 0.003490658503988666988 ) ;
#14303=DIRECTION ( 'NONE',  ( 0.000000000000000000, 0.000000000000000000, 1.000000000000000000 ) ) ;
#14304=EDGE_LOOP ( 'NONE', ( #3603, #105185, #36368, #124928 ) ) ;
#14305=DIRECTION ( 'NONE',  ( -0.000000000000000000, -1.000000000000000000, -0.000000000000000000 ) ) ;
#14306=ORIENTED_EDGE ( 'NONE', *, *, #65959, .F. ) ;
#14307=ORIENTED_EDGE ( 'NONE', *, *, #78669, .T. ) ;
#14308=ORIENTED_EDGE ( 'NONE', *, *, #26067, .T. ) ;
#14309=VERTEX_POINT ( 'NONE', #25093 ) ;
#14310=CONICAL_SURFACE ( 'NONE', #72913, 0.09999999999999982514, 0.003490658503988666988 ) ;
#14311=CARTESIAN_POINT ( 'NONE',  ( 1.049999999999952083, 2.500000000000000000, 6.841600689897072485 ) ) ;
#14312=FACE_BOUND ( 'NONE', #98129, .T. ) ;
#14313=DIRECTION ( 'NONE',  ( -0.000000000000000000, 1.000000000000000000, -0.000000000000000000 ) ) ;
#14314=AXIS2_PLACEMENT_3D ( 'NONE', #53949, #64403, #124621 ) ;
#14315=CIRCLE ( 'NONE', #125154, 0.06509327318403745899 ) ;
#14316=ORIENTED_EDGE ( 'NONE', *, *, #62439, .T. ) ;
#14317=DIRECTION ( 'NONE',  ( 0.000000000000000000, 1.000000000000000000, 0.000000000000000000 ) ) ;
#14318=DIRECTION ( 'NONE',  ( 0.000000000000000000, 0.000000000000000000, -1.000000000000000000 ) ) ;
#14319=ORIENTED_EDGE ( 'NONE', *, *, #53415, .T. ) ;
#14320=CARTESIAN_POINT ( 'NONE',  ( -5.000000000000023093, 2.500000000000000000, 0.6928203230275494784 ) ) ;
#14321=DIRECTION ( 'NONE',  ( 0.000000000000000000, 1.000000000000000000, 0.000000000000000000 ) ) ;
#14322=EDGE_CURVE ( 'NONE', #68325, #18847, #51702, .T. ) ;
#14323=ORIENTED_EDGE ( 'NONE', *, *, #90524, .F. ) ;
#14324=AXIS2_PLACEMENT_3D ( 'NONE', #65355, #2558, #13680 ) ;
#14325=DIRECTION ( 'NONE',  ( 0.000000000000000000, -0.000000000000000000, 1.000000000000000000 ) ) ;
#14326=DIRECTION ( 'NONE',  ( 0.000000000000000000, 1.000000000000000000, 0.000000000000000000 ) ) ;
#14327=ADVANCED_FACE ( 'NONE', ( #94466 ), #44749, .T. ) ;
#14328=ORIENTED_EDGE ( 'NONE', *, *, #77498, .T. ) ;
#14329=AXIS2_PLACEMENT_3D ( 'NONE', #100870, #87823, #127764 ) ;
#14330=CARTESIAN_POINT ( 'NONE',  ( 10.44999999999991047, 2.500000000000000000, -6.495190528383302464 ) ) ;
#14331=CIRCLE ( 'NONE', #127239, 0.06509327318403745899 ) ;
#14332=CARTESIAN_POINT ( 'NONE',  ( -7.100000000000013856, 2.500000000000000000, 3.537306695894645081 ) ) ;
#14333=CIRCLE ( 'NONE', #1828, 0.06509327318403745899 ) ;
#14334=DIRECTION ( 'NONE',  ( 0.000000000000000000, 0.000000000000000000, 1.000000000000000000 ) ) ;
#14335=EDGE_LOOP ( 'NONE', ( #112103, #29750 ) ) ;
#14336=EDGE_CURVE ( 'NONE', #103569, #116451, #60030, .T. ) ;
#14337=ORIENTED_EDGE ( 'NONE', *, *, #5394, .F. ) ;
#14338=EDGE_CURVE ( 'NONE', #104652, #118880, #55807, .T. ) ;
#14339=LINE ( 'NONE', #54283, #72364 ) ;
#14340=AXIS2_PLACEMENT_3D ( 'NONE', #115276, #98239, #125750 ) ;
#14341=VERTEX_POINT ( 'NONE', #44089 ) ;
#14342=DIRECTION ( 'NONE',  ( -0.000000000000000000, 1.000000000000000000, -0.000000000000000000 ) ) ;
#14343=CARTESIAN_POINT ( 'NONE',  ( -13.94999999999998685, 2.500000000000000000, -2.511473670974875727 ) ) ;
#14344=VECTOR ( 'NONE', #84420, 1000.000000000000000 ) ;
#14345=EDGE_LOOP ( 'NONE', ( #64424, #24627 ) ) ;
#14346=EDGE_CURVE ( 'NONE', #41508, #22099, #7767, .T. ) ;
#14347=CONICAL_SURFACE ( 'NONE', #104253, 0.09999999999999982514, 0.003490658503988666988 ) ;
#14348=DIRECTION ( 'NONE',  ( 0.000000000000000000, 0.000000000000000000, -1.000000000000000000 ) ) ;
#14349=DIRECTION ( 'NONE',  ( 0.000000000000000000, 0.000000000000000000, 1.000000000000000000 ) ) ;
#14350=CARTESIAN_POINT ( 'NONE',  ( 7.499999999999925393, 2.500000000000000000, -0.5928203230275541635 ) ) ;
#14351=DIRECTION ( 'NONE',  ( 0.000000000000000000, 0.000000000000000000, 1.000000000000000000 ) ) ;
#14352=EDGE_CURVE ( 'NONE', #25279, #102784, #112247, .T. ) ;
#14353=CARTESIAN_POINT ( 'NONE',  ( -10.60000000000000142, 2.500000000000000000, 4.083716857408421497 ) ) ;
#14354=CIRCLE ( 'NONE', #108448, 0.1000000000000002554 ) ;
#14355=ORIENTED_EDGE ( 'NONE', *, *, #55964, .F. ) ;
#14356=VERTEX_POINT ( 'NONE', #75474 ) ;
#14357=CARTESIAN_POINT ( 'NONE',  ( 4.149999999999941735, 2.500000000000000000, -5.702370205355749455 ) ) ;
#14358=CARTESIAN_POINT ( 'NONE',  ( -0.8500000000000386136, 12.50000000000000000, 5.802370205355744659 ) ) ;
#14359=DIRECTION ( 'NONE',  ( 0.000000000000000000, 1.000000000000000000, 0.000000000000000000 ) ) ;
#14360=ORIENTED_EDGE ( 'NONE', *, *, #66115, .T. ) ;
#14361=ORIENTED_EDGE ( 'NONE', *, *, #10557, .T. ) ;
#14362=ORIENTED_EDGE ( 'NONE', *, *, #11073, .F. ) ;
#14363=DIRECTION ( 'NONE',  ( 0.000000000000000000, 0.000000000000000000, 1.000000000000000000 ) ) ;
#14364=VECTOR ( 'NONE', #49634, 1000.000000000000000 ) ;
#14365=CARTESIAN_POINT ( 'NONE',  ( -3.643930204294122679E-14, 12.50000000000000000, 0.6277270498435143509 ) ) ;
#14366=DIRECTION ( 'NONE',  ( -0.000000000000000000, -1.000000000000000000, -0.000000000000000000 ) ) ;
#14368=CARTESIAN_POINT ( 'NONE',  ( 11.04999999999991189, 2.500000000000000000, -2.611473670974877592 ) ) ;
#14369=CARTESIAN_POINT ( 'NONE',  ( 9.599999999999914380, 2.500000000000000000, -5.022947341949754119 ) ) ;
#14370=LINE ( 'NONE', #22931, #38200 ) ;
#14371=CARTESIAN_POINT ( 'NONE',  ( 11.84999999999990372, 12.50000000000000000, 2.511473670974873507 ) ) ;
#14372=AXIS2_PLACEMENT_3D ( 'NONE', #114392, #126805, #37143 ) ;
#14373=CARTESIAN_POINT ( 'NONE',  ( -11.24999999999999822, 2.500000000000000000, 5.702370205355745014 ) ) ;
#14374=DIRECTION ( 'NONE',  ( 0.000000000000000000, 0.000000000000000000, 1.000000000000000000 ) ) ;
#14375=ORIENTED_EDGE ( 'NONE', *, *, #99412, .T. ) ;
#14376=EDGE_CURVE ( 'NONE', #78982, #24357, #89256, .T. ) ;
#14377=VECTOR ( 'NONE', #12147, 1000.000000000000000 ) ;
#14378=DIRECTION ( 'NONE',  ( -0.000000000000000000, -1.000000000000000000, -0.000000000000000000 ) ) ;
#14379=ORIENTED_EDGE ( 'NONE', *, *, #54875, .T. ) ;
#14380=EDGE_LOOP ( 'NONE', ( #71649, #115904 ) ) ;
#14381=EDGE_CURVE ( 'NONE', #6322, #36965, #22374, .T. ) ;
#14382=DIRECTION ( 'NONE',  ( 0.000000000000000000, 0.000000000000000000, -1.000000000000000000 ) ) ;
#14383=DIRECTION ( 'NONE',  ( 0.000000000000000000, 1.000000000000000000, 0.000000000000000000 ) ) ;
#14384=AXIS2_PLACEMENT_3D ( 'NONE', #40827, #89895, #98412 ) ;
#14385=CARTESIAN_POINT ( 'NONE',  ( -2.100000000000034284, 2.500000000000000000, 0.09999999999999761857 ) ) ;
#14386=EDGE_CURVE ( 'NONE', #50878, #74924, #126526, .T. ) ;
#14387=CARTESIAN_POINT ( 'NONE',  ( 1.649999999999951950, 12.50000000000000000, -7.122917578226816815 ) ) ;
#14388=AXIS2_PLACEMENT_3D ( 'NONE', #14434, #4597, #36032 ) ;
#14389=DIRECTION ( 'NONE',  ( 0.000000000000000000, 0.000000000000000000, 1.000000000000000000 ) ) ;
#14390=FACE_OUTER_BOUND ( 'NONE', #18638, .T. ) ;
#14391=CARTESIAN_POINT ( 'NONE',  ( 11.84999999999990372, 12.50000000000000000, 1.818653347947321475 ) ) ;
#14392=ORIENTED_EDGE ( 'NONE', *, *, #89579, .F. ) ;
#14393=CARTESIAN_POINT ( 'NONE',  ( -4.550000000000022915, 12.50000000000000000, -2.099970236277064473 ) ) ;
#14394=ADVANCED_FACE ( 'NONE', ( #25732 ), #3574, .T. ) ;
#14395=AXIS2_PLACEMENT_3D ( 'NONE', #60597, #40963, #71682 ) ;
#14396=ADVANCED_FACE ( 'NONE', ( #124592 ), #105602, .T. ) ;
#14398=LINE ( 'NONE', #104711, #72938 ) ;
#14399=VERTEX_POINT ( 'NONE', #13970 ) ;
#14400=ORIENTED_EDGE ( 'NONE', *, *, #25909, .T. ) ;
#14401=EDGE_CURVE ( 'NONE', #88713, #2945, #47496, .T. ) ;
#14402=VERTEX_POINT ( 'NONE', #98991 ) ;
#14403=AXIS2_PLACEMENT_3D ( 'NONE', #129317, #52028, #121398 ) ;
#14404=VERTEX_POINT ( 'NONE', #9968 ) ;
#14405=CARTESIAN_POINT ( 'NONE',  ( 10.39999999999991154, 2.500000000000000000, 3.537306695894645081 ) ) ;
#14406=CARTESIAN_POINT ( 'NONE',  ( 10.39999999999991154, 2.500000000000000000, -5.022947341949754119 ) ) ;
#14407=EDGE_CURVE ( 'NONE', #48905, #38438, #87185, .T. ) ;
#14408=CONICAL_SURFACE ( 'NONE', #29116, 0.1000000000000000056, 0.003490658503988666988 ) ;
#14409=CONICAL_SURFACE ( 'NONE', #87573, 0.09999999999999982514, 0.003490658503988666988 ) ;
#14410=EDGE_CURVE ( 'NONE', #120005, #16509, #76738, .T. ) ;
#14411=CARTESIAN_POINT ( 'NONE',  ( -3.550000000000028244, 12.50000000000000000, 2.511473670974873507 ) ) ;
#14412=CARTESIAN_POINT ( 'NONE',  ( 8.349999999999923261, 12.50000000000000000, 2.230156782645134950 ) ) ;
#14413=DIRECTION ( 'NONE',  ( 0.000000000000000000, -0.000000000000000000, 1.000000000000000000 ) ) ;
#14414=ORIENTED_EDGE ( 'NONE', *, *, #100341, .F. ) ;
#14415=CARTESIAN_POINT ( 'NONE',  ( -6.450000000000017941, 2.500000000000000000, -6.741600689897077281 ) ) ;
#14416=CARTESIAN_POINT ( 'NONE',  ( 2.299999999999946976, 12.50000000000000000, 4.611443907251934426 ) ) ;
#14417=CARTESIAN_POINT ( 'NONE',  ( -1.900000000000034994, 12.50000000000000000, -0.3464101615137783474 ) ) ;
#14418=ORIENTED_EDGE ( 'NONE', *, *, #76219, .F. ) ;
#14419=ORIENTED_EDGE ( 'NONE', *, *, #66682, .T. ) ;
#14420=ORIENTED_EDGE ( 'NONE', *, *, #215, .T. ) ;
#14421=AXIS2_PLACEMENT_3D ( 'NONE', #122058, #72315, #11443 ) ;
#14422=CARTESIAN_POINT ( 'NONE',  ( 2.299999999999946976, 2.500000000000000000, 4.676537180435972552 ) ) ;
#14423=CARTESIAN_POINT ( 'NONE',  ( 11.89999999999990443, 2.500000000000000000, -0.2464101615137782308 ) ) ;
#14424=CARTESIAN_POINT ( 'NONE',  ( -11.05000000000000249, 2.500000000000000000, -6.048780366869523029 ) ) ;
#14425=AXIS2_PLACEMENT_3D ( 'NONE', #14417, #96848, #85101 ) ;
#14426=CIRCLE ( 'NONE', #108532, 0.09999999999999982514 ) ;
#14427=ORIENTED_EDGE ( 'NONE', *, *, #48484, .F. ) ;
#14428=DIRECTION ( 'NONE',  ( 0.000000000000000000, 0.000000000000000000, 1.000000000000000000 ) ) ;
#14429=CARTESIAN_POINT ( 'NONE',  ( -12.69999999999999218, 2.500000000000000000, -0.2464101615137741230 ) ) ;
#14430=DIRECTION ( 'NONE',  ( 0.000000000000000000, 0.000000000000000000, 1.000000000000000000 ) ) ;
#14431=CARTESIAN_POINT ( 'NONE',  ( 9.599999999999914380, 12.50000000000000000, 5.088040615133786027 ) ) ;
#14432=AXIS2_PLACEMENT_3D ( 'NONE', #105713, #95889, #46138 ) ;
#14433=CIRCLE ( 'NONE', #93880, 0.1000000000000002554 ) ;
#14434=CARTESIAN_POINT ( 'NONE',  ( -9.800000000000006040, 2.500000000000000000, 4.676537180435972552 ) ) ;
#14435=EDGE_CURVE ( 'NONE', #123378, #52442, #108156, .T. ) ;
#14436=EDGE_LOOP ( 'NONE', ( #71460, #95093 ) ) ;
#14437=EDGE_LOOP ( 'NONE', ( #23274, #109808 ) ) ;
#14438=CARTESIAN_POINT ( 'NONE',  ( -9.800000000000007816, 2.500000000000000000, -4.083716857408422385 ) ) ;
#14439=DIRECTION ( 'NONE',  ( 0.000000000000000000, 0.000000000000000000, 1.000000000000000000 ) ) ;
#14440=AXIS2_PLACEMENT_3D ( 'NONE', #88525, #117312, #125869 ) ;
#14441=DIRECTION ( 'NONE',  ( 0.000000000000000000, 0.000000000000000000, -1.000000000000000000 ) ) ;
#14442=CARTESIAN_POINT ( 'NONE',  ( 11.24999999999990941, 12.50000000000000000, -1.472243186433550122 ) ) ;
#14443=CARTESIAN_POINT ( 'NONE',  ( -6.900000000000015454, 2.500000000000000000, 4.576537180435972019 ) ) ;
#14444=EDGE_CURVE ( 'NONE', #2289, #27095, #48608, .T. ) ;
#14445=VECTOR ( 'NONE', #44368, 1000.000000000000000 ) ;
#14446=VERTEX_POINT ( 'NONE', #27034 ) ;
#14447=VERTEX_POINT ( 'NONE', #47972 ) ;
#14448=CARTESIAN_POINT ( 'NONE',  ( 9.349999999999916156, 2.500000000000000000, -1.818653347947326138 ) ) ;
#14449=DIRECTION ( 'NONE',  ( 0.000000000000000000, 0.000000000000000000, -1.000000000000000000 ) ) ;
#14450=LINE ( 'NONE', #70976, #19376 ) ;
#14452=ORIENTED_EDGE ( 'NONE', *, *, #15132, .F. ) ;
#14453=CARTESIAN_POINT ( 'NONE',  ( -0.4000000000000404898, 2.500000000000000000, 4.922947341949748257 ) ) ;
#14454=DIRECTION ( 'NONE',  ( 0.000000000000000000, 0.000000000000000000, -1.000000000000000000 ) ) ;
#14455=AXIS2_PLACEMENT_3D ( 'NONE', #401, #128092, #69151 ) ;
#14456=ORIENTED_EDGE ( 'NONE', *, *, #120957, .T. ) ;
#14457=DIRECTION ( 'NONE',  ( -0.000000000000000000, -1.000000000000000000, -0.000000000000000000 ) ) ;
#14458=( BOUNDED_SURFACE ( )  B_SPLINE_SURFACE ( 2, 3, ( 
 ( #11515, #61272, #1683, #2994 ),
 ( #101834, #122129, #42944, #110983 ),
 ( #80909, #111659, #101192, #62569 ),
 ( #123395, #82856, #82197, #41653 ),
 ( #121456, #22644, #1048, #52096 ) ),
 .UNSPECIFIED., .F., .F., .F. ) 
 B_SPLINE_SURFACE_WITH_KNOTS ( ( 3, 2, 3 ),
 ( 4, 4 ),
 ( -0.1337713181301400378, 0.000000000000000000, 1.000000000000000000 ),
 ( -0.0002500000000000000052, 0.005250000000000000326 ),
 .UNSPECIFIED. ) 
 GEOMETRIC_REPRESENTATION_ITEM ( )  RATIONAL_B_SPLINE_SURFACE ( (
 ( 1.000000000000000000, 1.000000000000000000, 1.000000000000000000, 1.000000000000000000),
 ( 1.000000000000000000, 1.000000000000000000, 1.000000000000000000, 1.000000000000000000),
 ( 1.000000000000000000, 1.000000000000000000, 1.000000000000000000, 1.000000000000000000),
 ( 0.7071067811865475727, 0.7071067811865475727, 0.7071067811865475727, 0.7071067811865475727),
 ( 1.000000000000000000, 1.000000000000000000, 1.000000000000000000, 1.000000000000000000) ) ) 
 REPRESENTATION_ITEM ( '' )  SURFACE ( )  );
#14459=EDGE_LOOP ( 'NONE', ( #92361, #92682 ) ) ;
#14460=DIRECTION ( 'NONE',  ( 0.000000000000000000, -0.000000000000000000, 1.000000000000000000 ) ) ;
#14461=ORIENTED_EDGE ( 'NONE', *, *, #83070, .F. ) ;
#14462=DIRECTION ( 'NONE',  ( 0.000000000000000000, 0.000000000000000000, 1.000000000000000000 ) ) ;
#14463=DIRECTION ( 'NONE',  ( -0.000000000000000000, -1.000000000000000000, -0.000000000000000000 ) ) ;
#14464=ORIENTED_EDGE ( 'NONE', *, *, #60258, .T. ) ;
#14465=ORIENTED_EDGE ( 'NONE', *, *, #123776, .F. ) ;
#14468=AXIS2_PLACEMENT_3D ( 'NONE', #53213, #64301, #44032 ) ;
#14470=DIRECTION ( 'NONE',  ( 0.000000000000000000, 0.000000000000000000, -1.000000000000000000 ) ) ;
#14471=CARTESIAN_POINT ( 'NONE',  ( 8.549999999999918998, 2.500000000000000000, 6.941600689897073018 ) ) ;
#14472=CARTESIAN_POINT ( 'NONE',  ( 1.449999999999952216, 2.500000000000000000, 1.818653347947321475 ) ) ;
#14473=CARTESIAN_POINT ( 'NONE',  ( 5.399999999999934630, 2.500000000000000000, -0.6928203230275542523 ) ) ;
#14474=DIRECTION ( 'NONE',  ( -0.000000000000000000, -1.000000000000000000, -0.000000000000000000 ) ) ;
#14475=AXIS2_PLACEMENT_3D ( 'NONE', #51270, #70247, #110175 ) ;
#14476=ADVANCED_FACE ( 'NONE', ( #128473 ), #27650, .T. ) ;
#14477=EDGE_LOOP ( 'NONE', ( #13243, #68914 ) ) ;
#14478=EDGE_LOOP ( 'NONE', ( #98235, #33496, #89148, #6517 ) ) ;
#14479=DIRECTION ( 'NONE',  ( -0.000000000000000000, -1.000000000000000000, -0.000000000000000000 ) ) ;
#14480=AXIS2_PLACEMENT_3D ( 'NONE', #109063, #128095, #7656 ) ;
#14481=CONICAL_SURFACE ( 'NONE', #47970, 0.1000000000000002554, 0.003490658503988666988 ) ;
#14482=DIRECTION ( 'NONE',  ( 0.000000000000000000, 0.000000000000000000, -1.000000000000000000 ) ) ;
#14483=CARTESIAN_POINT ( 'NONE',  ( -14.79999999999998472, 12.50000000000000000, 0.3464101615137758494 ) ) ;
#14484=DIRECTION ( 'NONE',  ( 0.000000000000000000, 0.000000000000000000, -1.000000000000000000 ) ) ;
#14485=CIRCLE ( 'NONE', #1985, 0.06509327318403745899 ) ;
#14486=ORIENTED_EDGE ( 'NONE', *, *, #67206, .T. ) ;
#14487=ORIENTED_EDGE ( 'NONE', *, *, #126855, .T. ) ;
#14488=EDGE_CURVE ( 'NONE', #40728, #124471, #74676, .T. ) ;
#14489=FACE_BOUND ( 'NONE', #72417, .T. ) ;
#14490=ORIENTED_EDGE ( 'NONE', *, *, #64077, .F. ) ;
#14491=ADVANCED_FACE ( 'NONE', ( #117978 ), #62083, .T. ) ;
#14492=FACE_OUTER_BOUND ( 'NONE', #123804, .T. ) ;
#14493=DIRECTION ( 'NONE',  ( 0.000000000000000000, -0.000000000000000000, 1.000000000000000000 ) ) ;
#14494=EDGE_LOOP ( 'NONE', ( #68779, #88285, #114812, #43315 ) ) ;
#14495=DIRECTION ( 'NONE',  ( 0.000000000000000000, 1.000000000000000000, 0.000000000000000000 ) ) ;
#14496=VECTOR ( 'NONE', #100536, 1000.000000000000000 ) ;
#14497=CIRCLE ( 'NONE', #62652, 0.06509327318403745899 ) ;
#14498=CARTESIAN_POINT ( 'NONE',  ( -7.900000000000014566, 2.500000000000000000, -5.122947341949753763 ) ) ;
#14499=PLANE ( 'NONE',  #47259 ) ;
#14500=DIRECTION ( 'NONE',  ( -0.000000000000000000, -1.000000000000000000, -0.000000000000000000 ) ) ;
#14501=EDGE_CURVE ( 'NONE', #63883, #24530, #49267, .T. ) ;
#14502=CARTESIAN_POINT ( 'NONE',  ( 1.249999999999954259, 12.50000000000000000, -7.122917578226816815 ) ) ;
#14503=ADVANCED_FACE ( 'NONE', ( #107524 ), #127181, .T. ) ;
#14504=DIRECTION ( 'NONE',  ( 0.000000000000000000, 0.000000000000000000, 1.000000000000000000 ) ) ;
#14506=DIRECTION ( 'NONE',  ( 0.000000000000000000, -0.000000000000000000, 1.000000000000000000 ) ) ;
#14507=EDGE_CURVE ( 'NONE', #41590, #2959, #118488, .T. ) ;
#14508=DIRECTION ( 'NONE',  ( 0.000000000000000000, 0.000000000000000000, 1.000000000000000000 ) ) ;
#14509=VERTEX_POINT ( 'NONE', #128 ) ;
#14510=ORIENTED_EDGE ( 'NONE', *, *, #62119, .F. ) ;
#14511=EDGE_LOOP ( 'NONE', ( #29037, #7273 ) ) ;
#14512=LINE ( 'NONE', #85835, #70072 ) ;
#14513=VERTEX_POINT ( 'NONE', #89173 ) ;
#14514=DIRECTION ( 'NONE',  ( 0.000000000000000000, 0.000000000000000000, 1.000000000000000000 ) ) ;
#14515=AXIS2_PLACEMENT_3D ( 'NONE', #84695, #116087, #74883 ) ;
#14516=ORIENTED_EDGE ( 'NONE', *, *, #120229, .T. ) ;
#14517=EDGE_LOOP ( 'NONE', ( #69099, #82975 ) ) ;
#14518=EDGE_LOOP ( 'NONE', ( #89468, #16055, #27398, #84579 ) ) ;
#14519=CARTESIAN_POINT ( 'NONE',  ( -9.600000000000008527, 12.50000000000000000, -2.385244779468109755E-15 ) ) ;
#14520=CIRCLE ( 'NONE', #43802, 0.06509327318403745899 ) ;
#14521=AXIS2_PLACEMENT_3D ( 'NONE', #55481, #14869, #75748 ) ;
#14522=DIRECTION ( 'NONE',  ( 0.000000000000000000, 0.000000000000000000, 1.000000000000000000 ) ) ;
#14523=DIRECTION ( 'NONE',  ( 0.000000000000000000, 0.000000000000000000, 1.000000000000000000 ) ) ;
#14525=CARTESIAN_POINT ( 'NONE',  ( -9.600000000000006750, 12.50000000000000000, 3.572213422710607489 ) ) ;
#14526=ORIENTED_EDGE ( 'NONE', *, *, #110001, .F. ) ;
#14527=CONICAL_SURFACE ( 'NONE', #125269, 0.09999999999999982514, 0.003490658503988666988 ) ;
#14528=CIRCLE ( 'NONE', #58390, 0.1000000000000000056 ) ;
#14529=LINE ( 'NONE', #54466, #104067 ) ;
#14530=AXIS2_PLACEMENT_3D ( 'NONE', #115965, #36780, #16456 ) ;
#14531=EDGE_LOOP ( 'NONE', ( #72387, #101579, #9771, #36133 ) ) ;
#14532=AXIS2_PLACEMENT_3D ( 'NONE', #86329, #124343, #105344 ) ;
#14533=ORIENTED_EDGE ( 'NONE', *, *, #117521, .T. ) ;
#14534=EDGE_LOOP ( 'NONE', ( #56775, #100350, #4082, #12638 ) ) ;
#14535=CARTESIAN_POINT ( 'NONE',  ( -5.000000000000026645, 2.500000000000000000, -3.637306695894650055 ) ) ;
#14536=VERTEX_POINT ( 'NONE', #106858 ) ;
#14537=VERTEX_POINT ( 'NONE', #28975 ) ;
#14538=ORIENTED_EDGE ( 'NONE', *, *, #64835, .F. ) ;
#14539=VECTOR ( 'NONE', #106868, 1000.000000000000000 ) ;
#14540=DIRECTION ( 'NONE',  ( 0.000000000000000000, 0.000000000000000000, -1.000000000000000000 ) ) ;
#14541=VECTOR ( 'NONE', #27782, 1000.000000000000000 ) ;
#14542=DIRECTION ( 'NONE',  ( -0.000000000000000000, 1.000000000000000000, -0.000000000000000000 ) ) ;
#14543=CARTESIAN_POINT ( 'NONE',  ( 2.299999999999947864, 2.500000000000000000, 3.883716857408421319 ) ) ;
#14544=AXIS2_PLACEMENT_3D ( 'NONE', #127797, #127172, #8015 ) ;
#14545=DIRECTION ( 'NONE',  ( 0.000000000000000000, -0.000000000000000000, 1.000000000000000000 ) ) ;
#14546=DIRECTION ( 'NONE',  ( 0.000000000000000000, 1.000000000000000000, 0.000000000000000000 ) ) ;
#14547=EDGE_CURVE ( 'NONE', #997, #66180, #34778, .T. ) ;
#14548=CARTESIAN_POINT ( 'NONE',  ( 1.699999999999951994, 12.50000000000000000, -2.276824562219559311E-15 ) ) ;
#14549=ORIENTED_EDGE ( 'NONE', *, *, #107799, .T. ) ;
#14551=EDGE_CURVE ( 'NONE', #53518, #96649, #107916, .T. ) ;
#14552=FACE_OUTER_BOUND ( 'NONE', #126213, .T. ) ;
#14553=VERTEX_POINT ( 'NONE', #68876 ) ;
#14554=DIRECTION ( 'NONE',  ( 0.000000000000000000, 1.000000000000000000, 0.000000000000000000 ) ) ;
#14555=EDGE_LOOP ( 'NONE', ( #35303, #107684 ) ) ;
#14557=ADVANCED_FACE ( 'NONE', ( #8020 ), #76622, .T. ) ;
#14558=VECTOR ( 'NONE', #65505, 1000.000000000000000 ) ;
#14559=ADVANCED_FACE ( 'NONE', ( #3368 ), #112686, .T. ) ;
#14560=ORIENTED_EDGE ( 'NONE', *, *, #22353, .F. ) ;
#14561=ORIENTED_EDGE ( 'NONE', *, *, #69519, .T. ) ;
#14562=FACE_OUTER_BOUND ( 'NONE', #18435, .T. ) ;
#14563=CARTESIAN_POINT ( 'NONE',  ( 8.749999999999923617, 2.500000000000000000, -7.188010851410854052 ) ) ;
#14564=EDGE_CURVE ( 'NONE', #34866, #7578, #1301, .T. ) ;
#14565=EDGE_CURVE ( 'NONE', #124238, #55845, #45233, .T. ) ;
#14566=CARTESIAN_POINT ( 'NONE',  ( -6.249999999999984901, 2.500000000000000000, -2.165063509461101710 ) ) ;
#14567=EDGE_LOOP ( 'NONE', ( #96342, #5407 ) ) ;
#14568=LINE ( 'NONE', #66250, #105603 ) ;
#14569=EDGE_LOOP ( 'NONE', ( #122881, #65882, #68301, #81817 ) ) ;
#14570=CARTESIAN_POINT ( 'NONE',  ( 5.599999999999934808, 2.500000000000000000, -4.576537180435978236 ) ) ;
#14571=FACE_OUTER_BOUND ( 'NONE', #40006, .T. ) ;
#14572=LINE ( 'NONE', #123257, #85704 ) ;
#14573=DIRECTION ( 'NONE',  ( 0.000000000000000000, 1.000000000000000000, 0.000000000000000000 ) ) ;
#14574=EDGE_CURVE ( 'NONE', #73886, #6433, #64092, .T. ) ;
#14575=DIRECTION ( 'NONE',  ( 0.000000000000000000, -0.000000000000000000, 1.000000000000000000 ) ) ;
#14576=ORIENTED_EDGE ( 'NONE', *, *, #64689, .F. ) ;
#14577=CIRCLE ( 'NONE', #2056, 0.09999999999999982514 ) ;
#14578=VERTEX_POINT ( 'NONE', #102839 ) ;
#14579=CARTESIAN_POINT ( 'NONE',  ( -7.700000000000012612, 12.50000000000000000, 4.611443907251934426 ) ) ;
#14580=CARTESIAN_POINT ( 'NONE',  ( 2.499999999999947153, 12.50000000000000000, -3.637306695894650055 ) ) ;
#14581=VECTOR ( 'NONE', #86056, 1000.000000000000000 ) ;
#14582=CIRCLE ( 'NONE', #48063, 0.06509327318403745899 ) ;
#14583=CIRCLE ( 'NONE', #39676, 0.06509327318403745899 ) ;
#14585=DIRECTION ( 'NONE',  ( 0.000000000000000000, 0.000000000000000000, 1.000000000000000000 ) ) ;
#14586=DIRECTION ( 'NONE',  ( 0.000000000000000000, 0.000000000000000000, -1.000000000000000000 ) ) ;
#14587=CARTESIAN_POINT ( 'NONE',  ( -6.050000000000017586, 2.500000000000000000, 1.918653347947321564 ) ) ;
#14588=DIRECTION ( 'NONE',  ( -0.000000000000000000, -1.000000000000000000, -0.000000000000000000 ) ) ;
#14589=ORIENTED_EDGE ( 'NONE', *, *, #53991, .F. ) ;
#14590=AXIS2_PLACEMENT_3D ( 'NONE', #2180, #25052, #42120 ) ;
#14591=AXIS2_PLACEMENT_3D ( 'NONE', #47154, #118458, #77255 ) ;
#14592=CARTESIAN_POINT ( 'NONE',  ( 7.099999999999927702, 2.500000000000000000, -3.637306695894650055 ) ) ;
#14593=CARTESIAN_POINT ( 'NONE',  ( 4.599999999999937472, 2.500000000000000000, 0.5928203230275495006 ) ) ;
#14594=FACE_OUTER_BOUND ( 'NONE', #80746, .T. ) ;
#14595=ORIENTED_EDGE ( 'NONE', *, *, #103376, .T. ) ;
#14596=DIRECTION ( 'NONE',  ( -4.274815082592931898E-19, -0.9999939076577903929, -0.003490651415223739937 ) ) ;
#14597=EDGE_CURVE ( 'NONE', #83387, #123828, #49451, .T. ) ;
#14598=ORIENTED_EDGE ( 'NONE', *, *, #78079, .T. ) ;
#14599=LINE ( 'NONE', #34284, #44671 ) ;
#14600=ORIENTED_EDGE ( 'NONE', *, *, #4214, .T. ) ;
#14601=DIRECTION ( 'NONE',  ( 0.000000000000000000, 1.000000000000000000, 0.000000000000000000 ) ) ;
#14602=DIRECTION ( 'NONE',  ( 0.000000000000000000, 1.000000000000000000, 0.000000000000000000 ) ) ;
#14603=DIRECTION ( 'NONE',  ( -0.000000000000000000, 1.000000000000000000, -0.000000000000000000 ) ) ;
#14604=VERTEX_POINT ( 'NONE', #70182 ) ;
#14605=CIRCLE ( 'NONE', #39707, 0.06509327318403745899 ) ;
#14606=DIRECTION ( 'NONE',  ( 0.000000000000000000, 1.000000000000000000, 0.000000000000000000 ) ) ;
#14607=AXIS2_PLACEMENT_3D ( 'NONE', #27085, #99697, #48659 ) ;
#14608=CARTESIAN_POINT ( 'NONE',  ( -8.950000000000009948, 2.500000000000000000, -6.941600689897073018 ) ) ;
#14609=ORIENTED_EDGE ( 'NONE', *, *, #123504, .T. ) ;
#14610=AXIS2_PLACEMENT_3D ( 'NONE', #77329, #116599, #17081 ) ;
#14611=CARTESIAN_POINT ( 'NONE',  ( 10.39999999999991509, 12.50000000000000000, 0.6928203230275494784 ) ) ;
#14612=EDGE_LOOP ( 'NONE', ( #96484, #34652, #81617, #83569 ) ) ;
#14613=ORIENTED_EDGE ( 'NONE', *, *, #61064, .T. ) ;
#14614=LINE ( 'NONE', #53293, #113205 ) ;
#14615=CARTESIAN_POINT ( 'NONE',  ( -4.150000000000024336, 2.500000000000000000, -2.857883832488653741 ) ) ;
#14616=FACE_OUTER_BOUND ( 'NONE', #83764, .T. ) ;
#14617=VERTEX_POINT ( 'NONE', #2712 ) ;
#14618=VECTOR ( 'NONE', #31252, 1000.000000000000000 ) ;
#14620=DIRECTION ( 'NONE',  ( -4.274815082592931898E-19, -0.9999939076577903929, -0.003490651415223739937 ) ) ;
#14621=ORIENTED_EDGE ( 'NONE', *, *, #65101, .T. ) ;
#14622=CONICAL_SURFACE ( 'NONE', #31394, 0.09999999999999999167, 0.003490658503988666988 ) ;
#14623=FACE_OUTER_BOUND ( 'NONE', #114680, .T. ) ;
#14624=CARTESIAN_POINT ( 'NONE',  ( -13.14999999999999147, 12.50000000000000000, -2.511473670974875727 ) ) ;
#14625=AXIS2_PLACEMENT_3D ( 'NONE', #31534, #111357, #2055 ) ;
#14626=CARTESIAN_POINT ( 'NONE',  ( -15.39999999999998082, 12.50000000000000000, 0.6928203230275518099 ) ) ;
#14627=FACE_OUTER_BOUND ( 'NONE', #111432, .T. ) ;
#14628=DIRECTION ( 'NONE',  ( 0.000000000000000000, 0.000000000000000000, 1.000000000000000000 ) ) ;
#14629=VECTOR ( 'NONE', #46547, 1000.000000000000000 ) ;
#14630=CARTESIAN_POINT ( 'NONE',  ( 12.89999999999990088, 2.500000000000000000, 4.230127018922196669 ) ) ;
#14631=DIRECTION ( 'NONE',  ( -0.000000000000000000, 1.000000000000000000, -0.000000000000000000 ) ) ;
#14632=AXIS2_PLACEMENT_3D ( 'NONE', #56121, #55494, #115686 ) ;
#14633=EDGE_CURVE ( 'NONE', #29713, #128031, #20187, .T. ) ;
#14634=ORIENTED_EDGE ( 'NONE', *, *, #55525, .F. ) ;
#14635=ORIENTED_EDGE ( 'NONE', *, *, #49910, .F. ) ;
#14636=EDGE_LOOP ( 'NONE', ( #51257, #54418, #80668, #63802 ) ) ;
#14637=ORIENTED_EDGE ( 'NONE', *, *, #122149, .F. ) ;
#14638=AXIS2_PLACEMENT_3D ( 'NONE', #109301, #18340, #88353 ) ;
#14639=CARTESIAN_POINT ( 'NONE',  ( 3.549999999999940314, 12.50000000000000000, 6.906693963081109722 ) ) ;
#14640=CARTESIAN_POINT ( 'NONE',  ( 7.299999999999926104, 12.50000000000000000, 4.741630453620009789 ) ) ;
#14641=CARTESIAN_POINT ( 'NONE',  ( 7.899999999999923084, 2.500000000000000000, -0.5928203230275542746 ) ) ;
#14642=EDGE_LOOP ( 'NONE', ( #20808, #50642 ) ) ;
#14643=ADVANCED_FACE ( 'NONE', ( #53122 ), #126800, .T. ) ;
#14644=FACE_BOUND ( 'NONE', #29822, .T. ) ;
#14645=ADVANCED_FACE ( 'NONE', ( #101573 ), #32726, .T. ) ;
#14646=DIRECTION ( 'NONE',  ( -0.000000000000000000, -1.000000000000000000, -0.000000000000000000 ) ) ;
#14647=CARTESIAN_POINT ( 'NONE',  ( -2.100000000000033396, 2.500000000000000000, -0.5928203230275542746 ) ) ;
#14648=DIRECTION ( 'NONE',  ( -4.274815082592931898E-19, -0.9999939076577903929, -0.003490651415223739937 ) ) ;
#14649=CARTESIAN_POINT ( 'NONE',  ( 12.04999999999990834, 2.500000000000000000, -2.265063509461101798 ) ) ;
#14650=CARTESIAN_POINT ( 'NONE',  ( 3.149999999999946176, 2.500000000000000000, -6.248780366869526759 ) ) ;
#14651=EDGE_CURVE ( 'NONE', #106111, #111925, #122598, .T. ) ;
#14652=DIRECTION ( 'NONE',  ( 0.000000000000000000, 0.000000000000000000, 1.000000000000000000 ) ) ;
#14653=ADVANCED_FACE ( 'NONE', ( #72119 ), #57758, .T. ) ;
#14654=CARTESIAN_POINT ( 'NONE',  ( 0.6499999999999566125, 12.50000000000000000, -6.841600689897077814 ) ) ;
#14655=DIRECTION ( 'NONE',  ( 0.000000000000000000, 0.000000000000000000, 1.000000000000000000 ) ) ;
#14656=EDGE_CURVE ( 'NONE', #18715, #18830, #121203, .T. ) ;
#14657=CARTESIAN_POINT ( 'NONE',  ( 11.84999999999990372, 12.50000000000000000, 1.883746621131358934 ) ) ;
#14658=EDGE_CURVE ( 'NONE', #10004, #20333, #99614, .T. ) ;
#14659=EDGE_CURVE ( 'NONE', #126889, #11040, #3462, .T. ) ;
#14660=FACE_OUTER_BOUND ( 'NONE', #22143, .T. ) ;
#14661=ORIENTED_EDGE ( 'NONE', *, *, #13804, .F. ) ;
#14662=ORIENTED_EDGE ( 'NONE', *, *, #13497, .T. ) ;
#14663=VERTEX_POINT ( 'NONE', #20432 ) ;
#14664=ORIENTED_EDGE ( 'NONE', *, *, #122607, .T. ) ;
#14665=DIRECTION ( 'NONE',  ( 0.000000000000000000, 1.000000000000000000, 0.000000000000000000 ) ) ;
#14666=ORIENTED_EDGE ( 'NONE', *, *, #100403, .T. ) ;
#14667=AXIS2_PLACEMENT_3D ( 'NONE', #102458, #100513, #81530 ) ;
#14668=CARTESIAN_POINT ( 'NONE',  ( -0.8500000000000382805, 12.50000000000000000, -2.857883832488653741 ) ) ;
#14669=CONICAL_SURFACE ( 'NONE', #8414, 0.1000000000000000472, 0.003490658503988666988 ) ;
#14670=EDGE_LOOP ( 'NONE', ( #7732, #7586, #92325, #87026 ) ) ;
#14671=EDGE_CURVE ( 'NONE', #2125, #83526, #42006, .T. ) ;
#14672=ORIENTED_EDGE ( 'NONE', *, *, #42509, .T. ) ;
#14673=AXIS2_PLACEMENT_3D ( 'NONE', #29152, #108957, #80821 ) ;
#14674=CARTESIAN_POINT ( 'NONE',  ( 6.714630671517820559, -1.499999999999809708, 9.763603585529462947 ) ) ;
#14675=CARTESIAN_POINT ( 'NONE',  ( -7.500000000000015099, 2.500000000000000000, -5.022947341949754119 ) ) ;
#14676=FACE_OUTER_BOUND ( 'NONE', #89649, .T. ) ;
#14677=LINE ( 'NONE', #54604, #53842 ) ;
#14678=ORIENTED_EDGE ( 'NONE', *, *, #8606, .F. ) ;
#14679=ORIENTED_EDGE ( 'NONE', *, *, #57830, .F. ) ;
#14680=ORIENTED_EDGE ( 'NONE', *, *, #123776, .T. ) ;
#14681=FACE_OUTER_BOUND ( 'NONE', #70610, .T. ) ;
#14682=EDGE_LOOP ( 'NONE', ( #32200, #68385 ) ) ;
#14683=CARTESIAN_POINT ( 'NONE',  ( 3.349999999999941025, 2.500000000000000000, 7.088010851410848190 ) ) ;
#14684=VERTEX_POINT ( 'NONE', #62931 ) ;
#14685=ORIENTED_EDGE ( 'NONE', *, *, #72479, .F. ) ;
#14686=DIRECTION ( 'NONE',  ( 0.000000000000000000, 0.000000000000000000, 1.000000000000000000 ) ) ;
#14687=CARTESIAN_POINT ( 'NONE',  ( -13.54999999999999005, 12.50000000000000000, -1.883746621131361376 ) ) ;
#14688=CARTESIAN_POINT ( 'NONE',  ( -9.600000000000008527, 12.50000000000000000, 0.06509327318403504425 ) ) ;
#14689=DIRECTION ( 'NONE',  ( 0.000000000000000000, 0.000000000000000000, -1.000000000000000000 ) ) ;
#14690=DIRECTION ( 'NONE',  ( 0.000000000000000000, -0.9999939076577903929, 0.003490651415223739937 ) ) ;
#14691=EDGE_CURVE ( 'NONE', #84006, #49812, #11892, .T. ) ;
#14692=EDGE_LOOP ( 'NONE', ( #48349, #107094 ) ) ;
#14693=EDGE_CURVE ( 'NONE', #81036, #26833, #72422, .T. ) ;
#14694=DIRECTION ( 'NONE',  ( 0.000000000000000000, -0.9999939076577903929, 0.003490651415223739937 ) ) ;
#14695=AXIS2_PLACEMENT_3D ( 'NONE', #10507, #40657, #104686 ) ;
#14696=AXIS2_PLACEMENT_3D ( 'NONE', #101979, #42422, #82351 ) ;
#14697=ORIENTED_EDGE ( 'NONE', *, *, #23886, .F. ) ;
#14698=CARTESIAN_POINT ( 'NONE',  ( 87.50000000000002842, 5.708722954879577927, -4.899943752027914101 ) ) ;
#14699=EDGE_CURVE ( 'NONE', #80576, #53696, #93344, .T. ) ;
#14700=ORIENTED_EDGE ( 'NONE', *, *, #61244, .F. ) ;
#14701=CARTESIAN_POINT ( 'NONE',  ( -6.249999999999981348, 12.50000000000000000, 6.430097255199259010 ) ) ;
#14702=CARTESIAN_POINT ( 'NONE',  ( -1.250000000000001110, 2.500000000000000000, -2.165063509461101710 ) ) ;
#14703=DIRECTION ( 'NONE',  ( 0.000000000000000000, 0.000000000000000000, 1.000000000000000000 ) ) ;
#14704=ADVANCED_FACE ( 'NONE', ( #80652 ), #70357, .T. ) ;
#14705=DIRECTION ( 'NONE',  ( 0.000000000000000000, 1.000000000000000000, 0.000000000000000000 ) ) ;
#14706=ORIENTED_EDGE ( 'NONE', *, *, #110387, .T. ) ;
#14707=VECTOR ( 'NONE', #83684, 1000.000000000000000 ) ;
#14708=ADVANCED_FACE ( 'NONE', ( #65501 ), #11765, .T. ) ;
#14709=CARTESIAN_POINT ( 'NONE',  ( -13.74999999999998757, 2.500000000000000000, 1.572243186433549544 ) ) ;
#14710=ADVANCED_FACE ( 'NONE', ( #15748 ), #84932, .T. ) ;
#14711=EDGE_CURVE ( 'NONE', #107108, #30682, #53632, .T. ) ;
#14712=CARTESIAN_POINT ( 'NONE',  ( -4.350000000000027178, 2.500000000000000000, -6.841600689897077814 ) ) ;
#14713=EDGE_LOOP ( 'NONE', ( #95763, #59497, #116777, #90557 ) ) ;
#14714=ORIENTED_EDGE ( 'NONE', *, *, #14789, .F. ) ;
#14715=ORIENTED_EDGE ( 'NONE', *, *, #122852, .T. ) ;
#14716=CARTESIAN_POINT ( 'NONE',  ( 1.899999999999951283, 2.500000000000000000, 0.4464101615137736623 ) ) ;
#14717=CARTESIAN_POINT ( 'NONE',  ( 2.949999999999946887, 2.500000000000000000, -6.495190528383302464 ) ) ;
#14719=DIRECTION ( 'NONE',  ( 0.000000000000000000, 0.000000000000000000, 1.000000000000000000 ) ) ;
#14720=ADVANCED_FACE ( 'NONE', ( #74688 ), #74475, .T. ) ;
#14721=CONICAL_SURFACE ( 'NONE', #69016, 0.09999999999999982514, 0.003490658503988666988 ) ;
#14722=CARTESIAN_POINT ( 'NONE',  ( 17.10613367507962224, 2.036230694789155304, -5.376205058613481746 ) ) ;
#14723=CARTESIAN_POINT ( 'NONE',  ( -1.450000000000036371, 2.500000000000000000, 2.511473670974873507 ) ) ;
#14724=CIRCLE ( 'NONE', #4259, 0.06509327318403745899 ) ;
#14726=DIRECTION ( 'NONE',  ( 0.000000000000000000, 0.000000000000000000, -1.000000000000000000 ) ) ;
#14727=ORIENTED_EDGE ( 'NONE', *, *, #38522, .F. ) ;
#14728=DIRECTION ( 'NONE',  ( 0.000000000000000000, 0.000000000000000000, 1.000000000000000000 ) ) ;
#14730=CARTESIAN_POINT ( 'NONE',  ( -4.350000000000023626, 2.500000000000000000, 1.918653347947321564 ) ) ;
#14731=LINE ( 'NONE', #105054, #2062 ) ;
#14732=ORIENTED_EDGE ( 'NONE', *, *, #9950, .T. ) ;
#14734=FACE_OUTER_BOUND ( 'NONE', #38299, .T. ) ;
#14735=VERTEX_POINT ( 'NONE', #25567 ) ;
#14736=CARTESIAN_POINT ( 'NONE',  ( -10.60000000000000142, 2.500000000000000000, 3.983716857408420964 ) ) ;
#14737=EDGE_CURVE ( 'NONE', #32850, #31560, #83851, .T. ) ;
#14738=ORIENTED_EDGE ( 'NONE', *, *, #102751, .T. ) ;
#14739=VERTEX_POINT ( 'NONE', #63586 ) ;
#14740=DIRECTION ( 'NONE',  ( -0.000000000000000000, 1.000000000000000000, -0.000000000000000000 ) ) ;
#14741=CONICAL_SURFACE ( 'NONE', #117242, 0.1000000000000002554, 0.003490658503988666988 ) ;
#14742=AXIS2_PLACEMENT_3D ( 'NONE', #90039, #29850, #109706 ) ;
#14743=ORIENTED_EDGE ( 'NONE', *, *, #89732, .T. ) ;
#14744=CARTESIAN_POINT ( 'NONE',  ( 15.24415751722852086, 2.474878586408646441, -4.460068884075279350 ) ) ;
#14745=DIRECTION ( 'NONE',  ( 0.000000000000000000, 1.000000000000000000, 0.000000000000000000 ) ) ;
#14746=FACE_OUTER_BOUND ( 'NONE', #63807, .T. ) ;
#14747=ORIENTED_EDGE ( 'NONE', *, *, #87837, .T. ) ;
#14748=AXIS2_PLACEMENT_3D ( 'NONE', #57765, #7347, #97674 ) ;
#14749=FACE_BOUND ( 'NONE', #6346, .T. ) ;
#14750=CARTESIAN_POINT ( 'NONE',  ( -3.550000000000031797, 2.500000000000000000, -6.048780366869526581 ) ) ;
#14751=DIRECTION ( 'NONE',  ( -0.000000000000000000, 1.000000000000000000, -0.000000000000000000 ) ) ;
#14752=EDGE_LOOP ( 'NONE', ( #95595, #71011 ) ) ;
#14753=CONICAL_SURFACE ( 'NONE', #33666, 0.1000000000000002554, 0.003490658503988666988 ) ;
#14754=CARTESIAN_POINT ( 'NONE',  ( 2.099999999999949463, 2.500000000000000000, -3.537306695894649966 ) ) ;
#14755=ADVANCED_FACE ( 'NONE', ( #105443 ), #24297, .T. ) ;
#14756=CARTESIAN_POINT ( 'NONE',  ( -9.600000000000008527, 12.50000000000000000, 4.395220292106234439 ) ) ;
#14757=ORIENTED_EDGE ( 'NONE', *, *, #25210, .F. ) ;
#14759=ORIENTED_EDGE ( 'NONE', *, *, #65628, .F. ) ;
#14760=CARTESIAN_POINT ( 'NONE',  ( 15.59999999999988951, 2.500000000000000000, 0.3464101615137735735 ) ) ;
#14761=CARTESIAN_POINT ( 'NONE',  ( 4.913542845204887044, 2.499999999999490630, 9.942462991356222801 ) ) ;
#14762=CARTESIAN_POINT ( 'NONE',  ( 12.04999999999990479, 2.500000000000000000, 2.065063509461097624 ) ) ;
#14763=FACE_BOUND ( 'NONE', #115835, .T. ) ;
#14764=ORIENTED_EDGE ( 'NONE', *, *, #111177, .T. ) ;
#14766=LINE ( 'NONE', #5601, #128469 ) ;
#14767=DIRECTION ( 'NONE',  ( 0.000000000000000000, 0.000000000000000000, -1.000000000000000000 ) ) ;
#14768=DIRECTION ( 'NONE',  ( 0.000000000000000000, 0.000000000000000000, 1.000000000000000000 ) ) ;
#14769=DIRECTION ( 'NONE',  ( -4.274815082592931898E-19, -0.9999939076577903929, -0.003490651415223739937 ) ) ;
#14771=DIRECTION ( 'NONE',  ( 0.000000000000000000, 0.000000000000000000, 1.000000000000000000 ) ) ;
#14772=AXIS2_PLACEMENT_3D ( 'NONE', #95565, #103455, #83175 ) ;
#14773=CIRCLE ( 'NONE', #21062, 0.1000000000000002554 ) ;
#14774=DIRECTION ( 'NONE',  ( 0.000000000000000000, -0.9999939076577903929, 0.003490651415223739937 ) ) ;
#14775=EDGE_CURVE ( 'NONE', #31372, #88700, #61956, .T. ) ;
#14776=ORIENTED_EDGE ( 'NONE', *, *, #41068, .T. ) ;
#14777=EDGE_LOOP ( 'NONE', ( #97360, #96448, #42090, #18338 ) ) ;
#14778=ORIENTED_EDGE ( 'NONE', *, *, #87307, .T. ) ;
#14779=ORIENTED_EDGE ( 'NONE', *, *, #4938, .T. ) ;
#14780=VERTEX_POINT ( 'NONE', #34129 ) ;
#14781=CARTESIAN_POINT ( 'NONE',  ( -12.09999999999999432, 12.50000000000000000, 3.637306695894644726 ) ) ;
#14782=DIRECTION ( 'NONE',  ( -0.000000000000000000, -1.000000000000000000, -0.000000000000000000 ) ) ;
#14783=ORIENTED_EDGE ( 'NONE', *, *, #68147, .F. ) ;
#14784=FACE_BOUND ( 'NONE', #115359, .T. ) ;
#14785=CONICAL_SURFACE ( 'NONE', #104606, 0.1000000000000002554, 0.003490658503988666988 ) ;
#14786=CARTESIAN_POINT ( 'NONE',  ( -2.950000000000033484, 2.500000000000000000, -6.495190528383302464 ) ) ;
#14787=DIRECTION ( 'NONE',  ( 0.000000000000000000, 1.000000000000000000, 0.000000000000000000 ) ) ;
#14788=VERTEX_POINT ( 'NONE', #15085 ) ;
#14789=EDGE_CURVE ( 'NONE', #105063, #14247, #55684, .T. ) ;
#14790=CARTESIAN_POINT ( 'NONE',  ( 7.049999999999928768, 2.500000000000000000, 6.495190528383297135 ) ) ;
#14791=ADVANCED_FACE ( 'NONE', ( #106083 ), #3548, .T. ) ;
#14792=LINE ( 'NONE', #54736, #17684 ) ;
#14793=EDGE_CURVE ( 'NONE', #103547, #125357, #128970, .T. ) ;
#14794=FACE_OUTER_BOUND ( 'NONE', #44310, .T. ) ;
#14795=EDGE_CURVE ( 'NONE', #47117, #51312, #122677, .T. ) ;
#14796=ORIENTED_EDGE ( 'NONE', *, *, #9119, .F. ) ;
#14797=DIRECTION ( 'NONE',  ( 0.000000000000000000, 0.000000000000000000, 1.000000000000000000 ) ) ;
#14798=VERTEX_POINT ( 'NONE', #94311 ) ;
#14799=VECTOR ( 'NONE', #25238, 1000.000000000000000 ) ;
#14800=ADVANCED_FACE ( 'NONE', ( #85143 ), #80925, .T. ) ;
#14801=ORIENTED_EDGE ( 'NONE', *, *, #119379, .T. ) ;
#14802=ORIENTED_EDGE ( 'NONE', *, *, #66433, .T. ) ;
#14803=DIRECTION ( 'NONE',  ( 0.000000000000000000, 0.000000000000000000, 1.000000000000000000 ) ) ;
#14804=DIRECTION ( 'NONE',  ( 0.000000000000000000, 0.000000000000000000, 1.000000000000000000 ) ) ;
#14805=DIRECTION ( 'NONE',  ( 0.000000000000000000, -0.9999939076577903929, 0.003490651415223739937 ) ) ;
#14806=ORIENTED_EDGE ( 'NONE', *, *, #66418, .T. ) ;
#14807=EDGE_CURVE ( 'NONE', #88198, #7615, #24942, .T. ) ;
#14808=CARTESIAN_POINT ( 'NONE',  ( 4.848431875657850831, 2.499999999999999556, -8.943854603572997775 ) ) ;
#14809=AXIS2_PLACEMENT_3D ( 'NONE', #35253, #54863, #5122 ) ;
#14811=CARTESIAN_POINT ( 'NONE',  ( 5.849999999999933031, 2.500000000000000000, 7.288010851410849256 ) ) ;
#14812=EDGE_CURVE ( 'NONE', #95681, #93842, #125074, .T. ) ;
#14813=CARTESIAN_POINT ( 'NONE',  ( 6.849999999999927702, 2.500000000000000000, 1.918653347947321564 ) ) ;
#14814=CIRCLE ( 'NONE', #64999, 0.06509327318403745899 ) ;
#14816=CARTESIAN_POINT ( 'NONE',  ( 11.24999999999994316, 2.500000000000000000, -6.395190528383301931 ) ) ;
#14817=ORIENTED_EDGE ( 'NONE', *, *, #57080, .F. ) ;
#14819=DIRECTION ( 'NONE',  ( 0.000000000000000000, 1.000000000000000000, 0.000000000000000000 ) ) ;
#14820=EDGE_CURVE ( 'NONE', #3679, #59594, #110169, .T. ) ;
#14821=VERTEX_POINT ( 'NONE', #55687 ) ;
#14822=CARTESIAN_POINT ( 'NONE',  ( 7.099999999999928590, 2.500000000000000000, 3.537306695894645081 ) ) ;
#14823=ORIENTED_EDGE ( 'NONE', *, *, #20146, .T. ) ;
#14824=VERTEX_POINT ( 'NONE', #116536 ) ;
#14825=DIRECTION ( 'NONE',  ( 0.000000000000000000, 1.000000000000000000, 0.000000000000000000 ) ) ;
#14826=CARTESIAN_POINT ( 'NONE',  ( -7.100000000000013856, 2.500000000000000000, 3.737306695894644371 ) ) ;
#14827=DIRECTION ( 'NONE',  ( -0.000000000000000000, -1.000000000000000000, -0.000000000000000000 ) ) ;
#14828=DIRECTION ( 'NONE',  ( -4.274815082592931898E-19, -0.9999939076577903929, -0.003490651415223739937 ) ) ;
#14829=LINE ( 'NONE', #5026, #26702 ) ;
#14830=ORIENTED_EDGE ( 'NONE', *, *, #105595, .F. ) ;
#14832=DIRECTION ( 'NONE',  ( 0.000000000000000000, 1.000000000000000000, 0.000000000000000000 ) ) ;
#14833=DIRECTION ( 'NONE',  ( 0.000000000000000000, 1.000000000000000000, 0.000000000000000000 ) ) ;
#14834=CONICAL_SURFACE ( 'NONE', #19050, 0.1000000000000000472, 0.003490658503988666988 ) ;
#14835=DIRECTION ( 'NONE',  ( -0.000000000000000000, -1.000000000000000000, -0.000000000000000000 ) ) ;
#14836=EDGE_LOOP ( 'NONE', ( #119214, #127360 ) ) ;
#14837=ORIENTED_EDGE ( 'NONE', *, *, #53286, .F. ) ;
#14838=CONICAL_SURFACE ( 'NONE', #98469, 0.1000000000000000472, 0.003490658503988666988 ) ;
#14839=VECTOR ( 'NONE', #57875, 1000.000000000000000 ) ;
#14840=CARTESIAN_POINT ( 'NONE',  ( -6.050000000000022027, 2.500000000000000000, -1.918653347947326004 ) ) ;
#14841=VERTEX_POINT ( 'NONE', #17687 ) ;
#14842=DIRECTION ( 'NONE',  ( 0.000000000000000000, 0.000000000000000000, -1.000000000000000000 ) ) ;
#14843=AXIS2_PLACEMENT_3D ( 'NONE', #87045, #16353, #96865 ) ;
#14844=FACE_OUTER_BOUND ( 'NONE', #122753, .T. ) ;
#14845=EDGE_LOOP ( 'NONE', ( #67908, #105755, #105138, #9713 ) ) ;
#14846=FACE_OUTER_BOUND ( 'NONE', #31651, .T. ) ;
#14847=FACE_OUTER_BOUND ( 'NONE', #35619, .T. ) ;
#14848=CARTESIAN_POINT ( 'NONE',  ( 2.699999999999944666, 2.500000000000000000, 4.676537180435972552 ) ) ;
#14849=CONICAL_SURFACE ( 'NONE', #106898, 0.1000000000000002554, 0.003490658503988666988 ) ;
#14850=CARTESIAN_POINT ( 'NONE',  ( 0.4499999999999552136, 2.500000000000000000, 6.495190528383297135 ) ) ;
#14852=EDGE_CURVE ( 'NONE', #31487, #85147, #16045, .T. ) ;
#14853=DIRECTION ( 'NONE',  ( 0.000000000000000000, 0.000000000000000000, 1.000000000000000000 ) ) ;
#14855=ADVANCED_FACE ( 'NONE', ( #57632 ), #20274, .T. ) ;
#14856=EDGE_LOOP ( 'NONE', ( #42196, #40888, #100993, #102917 ) ) ;
#14857=ORIENTED_EDGE ( 'NONE', *, *, #12751, .T. ) ;
#14859=LINE ( 'NONE', #35196, #65774 ) ;
#14861=DIRECTION ( 'NONE',  ( 0.000000000000000000, 1.000000000000000000, 0.000000000000000000 ) ) ;
#14862=EDGE_CURVE ( 'NONE', #82663, #30237, #47166, .T. ) ;
#14863=DIRECTION ( 'NONE',  ( -0.000000000000000000, -1.000000000000000000, -0.000000000000000000 ) ) ;
#14864=AXIS2_PLACEMENT_3D ( 'NONE', #117695, #126906, #38548 ) ;
#14865=DIRECTION ( 'NONE',  ( 0.000000000000000000, 1.000000000000000000, 0.000000000000000000 ) ) ;
#14866=DIRECTION ( 'NONE',  ( 0.000000000000000000, 0.000000000000000000, -1.000000000000000000 ) ) ;
#14867=DIRECTION ( 'NONE',  ( 0.000000000000000000, 0.000000000000000000, 1.000000000000000000 ) ) ;
#14868=CARTESIAN_POINT ( 'NONE',  ( -12.49999999999999467, 12.50000000000000000, -3.572213422710609709 ) ) ;
#14869=DIRECTION ( 'NONE',  ( 0.000000000000000000, 1.000000000000000000, 0.000000000000000000 ) ) ;
#14870=AXIS2_PLACEMENT_3D ( 'NONE', #37297, #97492, #18280 ) ;
#14871=ORIENTED_EDGE ( 'NONE', *, *, #96525, .T. ) ;
#14872=EDGE_LOOP ( 'NONE', ( #45782, #50244, #91802, #34045 ) ) ;
#14873=VERTEX_POINT ( 'NONE', #97541 ) ;
#14874=ORIENTED_EDGE ( 'NONE', *, *, #50573, .F. ) ;
#14875=CARTESIAN_POINT ( 'NONE',  ( -2.499999999999996003, 2.500000000000000000, -4.430127018922202176 ) ) ;
#14876=DIRECTION ( 'NONE',  ( -0.000000000000000000, -1.000000000000000000, -0.000000000000000000 ) ) ;
#14877=CARTESIAN_POINT ( 'NONE',  ( 6.249999999999934275, 2.500000000000000000, -7.288010851410854585 ) ) ;
#14878=AXIS2_PLACEMENT_3D ( 'NONE', #64831, #106052, #4590 ) ;
#14879=AXIS2_PLACEMENT_3D ( 'NONE', #120353, #60156, #100062 ) ;
#14880=EDGE_LOOP ( 'NONE', ( #73963, #96755 ) ) ;
#14881=DIRECTION ( 'NONE',  ( 0.000000000000000000, 1.000000000000000000, 0.000000000000000000 ) ) ;
#14882=DIRECTION ( 'NONE',  ( 0.000000000000000000, 0.000000000000000000, 1.000000000000000000 ) ) ;
#14883=DIRECTION ( 'NONE',  ( 0.000000000000000000, 0.000000000000000000, 1.000000000000000000 ) ) ;
#14884=ORIENTED_EDGE ( 'NONE', *, *, #57969, .F. ) ;
#14885=DIRECTION ( 'NONE',  ( 0.000000000000000000, 0.000000000000000000, 1.000000000000000000 ) ) ;
#14886=CIRCLE ( 'NONE', #2378, 0.1000000000000000472 ) ;
#14887=VERTEX_POINT ( 'NONE', #68726 ) ;
#14888=AXIS2_PLACEMENT_3D ( 'NONE', #37669, #118792, #127967 ) ;
#14889=EDGE_LOOP ( 'NONE', ( #89922, #83309 ) ) ;
#14890=ORIENTED_EDGE ( 'NONE', *, *, #50963, .T. ) ;
#14891=CIRCLE ( 'NONE', #63053, 0.09999999999999982514 ) ;
#14893=DIRECTION ( 'NONE',  ( 0.000000000000000000, 0.000000000000000000, -1.000000000000000000 ) ) ;
#14894=AXIS2_PLACEMENT_3D ( 'NONE', #28655, #108481, #118950 ) ;
#14895=CARTESIAN_POINT ( 'NONE',  ( 0.5999999999999621192, 2.500000000000000000, 0.4464101615137758272 ) ) ;
#14896=DIRECTION ( 'NONE',  ( -0.000000000000000000, 1.000000000000000000, -0.000000000000000000 ) ) ;
#14897=DIRECTION ( 'NONE',  ( 0.000000000000000000, 0.000000000000000000, 1.000000000000000000 ) ) ;
#14898=ORIENTED_EDGE ( 'NONE', *, *, #70668, .F. ) ;
#14899=AXIS2_PLACEMENT_3D ( 'NONE', #101600, #63609, #11915 ) ;
#14900=AXIS2_PLACEMENT_3D ( 'NONE', #96019, #6318, #8270 ) ;
#14901=CARTESIAN_POINT ( 'NONE',  ( 15.19999999999989271, 12.50000000000000000, -0.3464101615137783474 ) ) ;
#14902=EDGE_CURVE ( 'NONE', #31023, #63981, #60013, .T. ) ;
#14903=EDGE_LOOP ( 'NONE', ( #90595, #63160, #58820, #2268 ) ) ;
#14904=CARTESIAN_POINT ( 'NONE',  ( -0.8500000000000390576, 2.500000000000000000, -6.495190528383302464 ) ) ;
#14905=DIRECTION ( 'NONE',  ( -4.274815082592931898E-19, -0.9999939076577903929, -0.003490651415223739937 ) ) ;
#14906=DIRECTION ( 'NONE',  ( 0.000000000000000000, 0.000000000000000000, 1.000000000000000000 ) ) ;
#14907=DIRECTION ( 'NONE',  ( 0.000000000000000000, -0.9999939076577903929, 0.003490651415223739937 ) ) ;
#14908=EDGE_CURVE ( 'NONE', #89282, #111058, #53721, .T. ) ;
#14909=ORIENTED_EDGE ( 'NONE', *, *, #41056, .T. ) ;
#14910=ORIENTED_EDGE ( 'NONE', *, *, #126436, .F. ) ;
#14911=EDGE_LOOP ( 'NONE', ( #46141, #8446, #129296, #29986 ) ) ;
#14912=CARTESIAN_POINT ( 'NONE',  ( -8.749999999999971578, 2.500000000000000000, 6.595190528383296780 ) ) ;
#14913=CARTESIAN_POINT ( 'NONE',  ( -10.40000000000000213, 12.50000000000000000, -0.6277270498435166823 ) ) ;
#14915=CARTESIAN_POINT ( 'NONE',  ( -12.09999999999999609, 2.500000000000000000, -0.6928203230275501445 ) ) ;
#14916=FACE_BOUND ( 'NONE', #34306, .T. ) ;
#14917=CARTESIAN_POINT ( 'NONE',  ( -0.8500000000000390576, 12.50000000000000000, -6.495190528383302464 ) ) ;
#14918=CARTESIAN_POINT ( 'NONE',  ( 7.099999999999926814, 2.500000000000000000, -0.6928203230275541413 ) ) ;
#14919=DIRECTION ( 'NONE',  ( 0.000000000000000000, 1.000000000000000000, 0.000000000000000000 ) ) ;
#14920=AXIS2_PLACEMENT_3D ( 'NONE', #30113, #41860, #109951 ) ;
#14921=CIRCLE ( 'NONE', #117423, 0.06509327318403745899 ) ;
#14923=CONICAL_SURFACE ( 'NONE', #50544, 0.1000000000000002554, 0.003490658503988666988 ) ;
#14924=DIRECTION ( 'NONE',  ( 0.000000000000000000, 0.000000000000000000, 1.000000000000000000 ) ) ;
#14925=CARTESIAN_POINT ( 'NONE',  ( -1.050000000000038236, 12.50000000000000000, -6.148780366869526226 ) ) ;
#14926=ORIENTED_EDGE ( 'NONE', *, *, #120422, .F. ) ;
#14927=DIRECTION ( 'NONE',  ( 0.000000000000000000, 0.000000000000000000, 1.000000000000000000 ) ) ;
#14928=AXIS2_PLACEMENT_3D ( 'NONE', #116263, #43697, #94060 ) ;
#14929=EDGE_CURVE ( 'NONE', #48260, #79022, #128318, .T. ) ;
#14931=EDGE_LOOP ( 'NONE', ( #118999, #104730, #51864, #56684 ) ) ;
#14932=EDGE_LOOP ( 'NONE', ( #114353, #114710, #47308, #38871 ) ) ;
#14933=ORIENTED_EDGE ( 'NONE', *, *, #110387, .F. ) ;
#14934=CIRCLE ( 'NONE', #127837, 0.1000000000000002554 ) ;
#14935=CARTESIAN_POINT ( 'NONE',  ( -8.350000000000012079, 2.500000000000000000, 2.757883832488649656 ) ) ;
#14936=FACE_BOUND ( 'NONE', #77908, .T. ) ;
#14937=DIRECTION ( 'NONE',  ( 0.000000000000000000, -0.9999939076577903929, 0.003490651415223739937 ) ) ;
#14938=ADVANCED_FACE ( 'NONE', ( #88349 ), #26876, .T. ) ;
#14939=ORIENTED_EDGE ( 'NONE', *, *, #32757, .T. ) ;
#14940=ADVANCED_FACE ( 'NONE', ( #86429 ), #70453, .T. ) ;
#14941=CARTESIAN_POINT ( 'NONE',  ( 48.83465639036802486, 3.619824997320591820, 4.313881469043760575 ) ) ;
#14942=ADVANCED_FACE ( 'NONE', ( #79213 ), #45334, .T. ) ;
#14943=CARTESIAN_POINT ( 'NONE',  ( -11.44999999999999751, 12.50000000000000000, -6.841600689897074261 ) ) ;
#14944=ADVANCED_FACE ( 'NONE', ( #49113 ), #30764, .T. ) ;
#14945=EDGE_CURVE ( 'NONE', #92060, #3076, #118466, .T. ) ;
#14946=EDGE_LOOP ( 'NONE', ( #57425, #15279 ) ) ;
#14947=DIRECTION ( 'NONE',  ( 0.000000000000000000, -0.000000000000000000, 1.000000000000000000 ) ) ;
#14948=DIRECTION ( 'NONE',  ( 0.000000000000000000, 0.000000000000000000, 1.000000000000000000 ) ) ;
#14949=ADVANCED_FACE ( 'NONE', ( #89025 ), #114263, .T. ) ;
#14950=ORIENTED_EDGE ( 'NONE', *, *, #45039, .T. ) ;
#14951=FACE_OUTER_BOUND ( 'NONE', #48685, .T. ) ;
#14952=ADVANCED_FACE ( 'NONE', ( #77894 ), #47465, .T. ) ;
#14953=DIRECTION ( 'NONE',  ( -0.000000000000000000, -1.000000000000000000, -0.000000000000000000 ) ) ;
#14954=CIRCLE ( 'NONE', #58824, 0.06509327318403745899 ) ;
#14955=CONICAL_SURFACE ( 'NONE', #25434, 0.1000000000000000472, 0.003490658503988666988 ) ;
#14956=ADVANCED_FACE ( 'NONE', ( #68079 ), #49536, .T. ) ;
#14957=EDGE_LOOP ( 'NONE', ( #80212, #110968 ) ) ;
#14958=FACE_OUTER_BOUND ( 'NONE', #72790, .T. ) ;
#14959=EDGE_CURVE ( 'NONE', #9531, #34777, #78791, .T. ) ;
#14960=DIRECTION ( 'NONE',  ( 0.000000000000000000, 0.000000000000000000, -1.000000000000000000 ) ) ;
#14961=CARTESIAN_POINT ( 'NONE',  ( 14.54999999999989591, 2.500000000000000000, 2.065063509461097624 ) ) ;
#14962=ORIENTED_EDGE ( 'NONE', *, *, #38950, .F. ) ;
#14963=VERTEX_POINT ( 'NONE', #60849 ) ;
#14964=DIRECTION ( 'NONE',  ( 0.000000000000000000, 1.000000000000000000, 0.000000000000000000 ) ) ;
#14965=CONICAL_SURFACE ( 'NONE', #79757, 0.1000000000000002554, 0.003490658503988666988 ) ;
#14966=EDGE_CURVE ( 'NONE', #12831, #99549, #110588, .T. ) ;
#14967=VERTEX_POINT ( 'NONE', #30121 ) ;
#14968=PLANE ( 'NONE',  #63728 ) ;
#14969=CONICAL_SURFACE ( 'NONE', #96552, 0.09999999999999982514, 0.003490658503988666988 ) ;
#14970=DIRECTION ( 'NONE',  ( -0.000000000000000000, 1.000000000000000000, -0.000000000000000000 ) ) ;
#14971=CONICAL_SURFACE ( 'NONE', #121606, 0.09999999999999982514, 0.003490658503988666988 ) ;
#14972=ORIENTED_EDGE ( 'NONE', *, *, #106059, .T. ) ;
#14973=VECTOR ( 'NONE', #50191, 1000.000000000000000 ) ;
#14974=AXIS2_PLACEMENT_3D ( 'NONE', #25616, #74737, #83276 ) ;
#14976=DIRECTION ( 'NONE',  ( 0.000000000000000000, 0.000000000000000000, -1.000000000000000000 ) ) ;
#14977=DIRECTION ( 'NONE',  ( 0.000000000000000000, 1.000000000000000000, 0.000000000000000000 ) ) ;
#14978=( BOUNDED_SURFACE ( )  B_SPLINE_SURFACE ( 3, 2, ( 
 ( #119151, #37385, #58318 ),
 ( #127051, #76653, #116563 ),
 ( #77291, #117183, #98214 ),
 ( #89054, #17712, #70056 ) ),
 .UNSPECIFIED., .F., .F., .F. ) 
 B_SPLINE_SURFACE_WITH_KNOTS ( ( 4, 4 ),
 ( 3, 3 ),
 ( 0.02228103309872373275, 0.02393870366795243856 ),
 ( 0.000000000000000000, 1.000000000000000000 ),
 .UNSPECIFIED. ) 
 GEOMETRIC_REPRESENTATION_ITEM ( )  RATIONAL_B_SPLINE_SURFACE ( (
 ( 1.000000000000000000, 0.9066952437723005964, 1.000000000000000000),
 ( 1.000000000000000000, 0.9065452688549086036, 1.000000000000000000),
 ( 1.000000000000000000, 0.9065452844449171099, 1.000000000000000000),
 ( 1.000000000000000000, 0.9066952434955798390, 1.000000000000000000) ) ) 
 REPRESENTATION_ITEM ( '' )  SURFACE ( )  );
#14979=CARTESIAN_POINT ( 'NONE',  ( 9.999999999999911182, 2.500000000000000000, 5.122947341949749323 ) ) ;
#14980=CARTESIAN_POINT ( 'NONE',  ( -7.950000000000012612, 12.50000000000000000, 2.165063509461097713 ) ) ;
#14981=AXIS2_PLACEMENT_3D ( 'NONE', #101875, #21373, #63236 ) ;
#14982=ORIENTED_EDGE ( 'NONE', *, *, #56022, .F. ) ;
#14984=AXIS2_PLACEMENT_3D ( 'NONE', #87230, #78741, #36870 ) ;
#14985=ORIENTED_EDGE ( 'NONE', *, *, #121339, .T. ) ;
#14986=FACE_OUTER_BOUND ( 'NONE', #19590, .T. ) ;
#14987=CARTESIAN_POINT ( 'NONE',  ( -5.000000000000022204, 12.50000000000000000, -0.6277270498435166823 ) ) ;
#14988=CONICAL_SURFACE ( 'NONE', #63139, 0.1000000000000002554, 0.003490658503988666988 ) ;
#14989=AXIS2_PLACEMENT_3D ( 'NONE', #125775, #44026, #65581 ) ;
#14990=CIRCLE ( 'NONE', #42227, 0.09999999999999982514 ) ;
#14991=CARTESIAN_POINT ( 'NONE',  ( 8.949999999999917577, 12.50000000000000000, 6.083687093685482772 ) ) ;
#14992=ORIENTED_EDGE ( 'NONE', *, *, #82605, .T. ) ;
#14993=ORIENTED_EDGE ( 'NONE', *, *, #55470, .T. ) ;
#14994=ORIENTED_EDGE ( 'NONE', *, *, #74001, .T. ) ;
#14995=DIRECTION ( 'NONE',  ( 0.000000000000000000, -0.9999939076577903929, 0.003490651415223739937 ) ) ;
#14996=CIRCLE ( 'NONE', #79778, 0.06509327318403745899 ) ;
#14997=LINE ( 'NONE', #95530, #65315 ) ;
#14998=LINE ( 'NONE', #35327, #122894 ) ;
#14999=CARTESIAN_POINT ( 'NONE',  ( 3.349999999999941025, 2.500000000000000000, 7.288010851410849256 ) ) ;
#15000=VECTOR ( 'NONE', #111392, 1000.000000000000000 ) ;
#15001=CARTESIAN_POINT ( 'NONE',  ( -7.700000000000016165, 2.500000000000000000, 0.4464101615137735513 ) ) ;
#15002=CARTESIAN_POINT ( 'NONE',  ( 9.999999999999912959, 12.50000000000000000, -5.022947341949754119 ) ) ;
#15003=DIRECTION ( 'NONE',  ( -0.000000000000000000, -1.000000000000000000, -0.000000000000000000 ) ) ;
#15004=CARTESIAN_POINT ( 'NONE',  ( 3.149999999999946176, 2.500000000000000000, -2.511473670974877948 ) ) ;
#15005=B_SPLINE_CURVE_WITH_KNOTS ( 'NONE', 3,
 ( #727, #60327, #58389, #47919, #89760, #88458, #90384, #38761, #29554, #117925 ),
 .UNSPECIFIED., .F., .F.,
 ( 4, 2, 2, 2, 4 ),
 ( 0.003751885956794874175, 0.02035553200375762178, 0.03695917805072037460, 0.05356282409768312047, 0.07016647014464587329 ),
 .UNSPECIFIED. ) ;
#15006=DIRECTION ( 'NONE',  ( 0.000000000000000000, 1.000000000000000000, 0.000000000000000000 ) ) ;
#15007=ORIENTED_EDGE ( 'NONE', *, *, #22573, .F. ) ;
#15008=EDGE_CURVE ( 'NONE', #24288, #3310, #9812, .T. ) ;
#15009=ADVANCED_FACE ( 'NONE', ( #99496 ), #39083, .T. ) ;
#15010=DIRECTION ( 'NONE',  ( -0.000000000000000000, 1.000000000000000000, -0.000000000000000000 ) ) ;
#15011=EDGE_LOOP ( 'NONE', ( #127142, #24221, #124261, #78270 ) ) ;
#15012=ORIENTED_EDGE ( 'NONE', *, *, #35686, .F. ) ;
#15013=DIRECTION ( 'NONE',  ( 0.000000000000000000, 0.000000000000000000, -1.000000000000000000 ) ) ;
#15014=DIRECTION ( 'NONE',  ( 0.000000000000000000, 0.000000000000000000, -1.000000000000000000 ) ) ;
#15015=DIRECTION ( 'NONE',  ( 0.000000000000000000, 0.000000000000000000, 1.000000000000000000 ) ) ;
#15017=DIRECTION ( 'NONE',  ( -0.000000000000000000, 1.000000000000000000, -0.000000000000000000 ) ) ;
#15018=DIRECTION ( 'NONE',  ( 0.000000000000000000, -0.000000000000000000, 1.000000000000000000 ) ) ;
#15019=AXIS2_PLACEMENT_3D ( 'NONE', #14145, #103837, #84178 ) ;
#15020=CARTESIAN_POINT ( 'NONE',  ( -6.450000000000014388, 12.50000000000000000, 6.148780366869520897 ) ) ;
#15021=ORIENTED_EDGE ( 'NONE', *, *, #50913, .T. ) ;
#15022=CARTESIAN_POINT ( 'NONE',  ( 4.999999999999935163, 2.500000000000000000, 0.6928203230275494784 ) ) ;
#15023=CIRCLE ( 'NONE', #10905, 0.09999999999999982514 ) ;
#15024=DIRECTION ( 'NONE',  ( -0.000000000000000000, -1.000000000000000000, -0.000000000000000000 ) ) ;
#15025=ORIENTED_EDGE ( 'NONE', *, *, #3449, .F. ) ;
#15026=CONICAL_SURFACE ( 'NONE', #90350, 0.1000000000000000056, 0.003490658503988666988 ) ;
#15027=ORIENTED_EDGE ( 'NONE', *, *, #60916, .F. ) ;
#15028=CIRCLE ( 'NONE', #115375, 0.06509327318403745899 ) ;
#15029=ORIENTED_EDGE ( 'NONE', *, *, #21019, .T. ) ;
#15030=AXIS2_PLACEMENT_3D ( 'NONE', #2946, #71036, #99857 ) ;
#15031=AXIS2_PLACEMENT_3D ( 'NONE', #57108, #67556, #77400 ) ;
#15032=ORIENTED_EDGE ( 'NONE', *, *, #118281, .F. ) ;
#15033=CARTESIAN_POINT ( 'NONE',  ( 8.099999999999923261, 2.500000000000000000, -4.576537180435978236 ) ) ;
#15034=DIRECTION ( 'NONE',  ( 0.000000000000000000, -0.000000000000000000, 1.000000000000000000 ) ) ;
#15035=DIRECTION ( 'NONE',  ( -0.000000000000000000, 1.000000000000000000, -0.000000000000000000 ) ) ;
#15036=DIRECTION ( 'NONE',  ( 0.000000000000000000, 0.000000000000000000, 1.000000000000000000 ) ) ;
#15037=CARTESIAN_POINT ( 'NONE',  ( -10.40000000000000391, 2.500000000000000000, -3.537306695894645969 ) ) ;
#15038=EDGE_LOOP ( 'NONE', ( #120793, #121108 ) ) ;
#15039=CARTESIAN_POINT ( 'NONE',  ( 10.64999999999991331, 2.500000000000000000, -2.511473670974877948 ) ) ;
#15040=CARTESIAN_POINT ( 'NONE',  ( 6.849999999999929479, 2.500000000000000000, -1.718653347947326049 ) ) ;
#15041=DIRECTION ( 'NONE',  ( 0.000000000000000000, 0.000000000000000000, -1.000000000000000000 ) ) ;
#15042=EDGE_CURVE ( 'NONE', #90838, #110412, #95486, .T. ) ;
#15043=ORIENTED_EDGE ( 'NONE', *, *, #5543, .F. ) ;
#15044=ORIENTED_EDGE ( 'NONE', *, *, #82837, .F. ) ;
#15045=ORIENTED_EDGE ( 'NONE', *, *, #30758, .T. ) ;
#15046=CARTESIAN_POINT ( 'NONE',  ( -1.450000000000035039, 2.500000000000000000, -2.511473670974877948 ) ) ;
#15047=PLANE ( 'NONE',  #73867 ) ;
#15048=AXIS2_PLACEMENT_3D ( 'NONE', #4918, #3013, #33128 ) ;
#15049=DIRECTION ( 'NONE',  ( 0.000000000000000000, 1.000000000000000000, 0.000000000000000000 ) ) ;
#15050=EDGE_CURVE ( 'NONE', #85840, #25440, #109957, .T. ) ;
#15051=ORIENTED_EDGE ( 'NONE', *, *, #122780, .T. ) ;
#15052=DIRECTION ( 'NONE',  ( -0.000000000000000000, -1.000000000000000000, -0.000000000000000000 ) ) ;
#15053=LINE ( 'NONE', #65471, #1424 ) ;
#15055=DIRECTION ( 'NONE',  ( 0.000000000000000000, 0.000000000000000000, -1.000000000000000000 ) ) ;
#15056=EDGE_CURVE ( 'NONE', #51917, #43890, #55782, .T. ) ;
#15057=LINE ( 'NONE', #94290, #26886 ) ;
#15058=CIRCLE ( 'NONE', #35931, 0.06509327318403741736 ) ;
#15059=VECTOR ( 'NONE', #93792, 1000.000000000000000 ) ;
#15060=ORIENTED_EDGE ( 'NONE', *, *, #18086, .T. ) ;
#15061=DIRECTION ( 'NONE',  ( 0.000000000000000000, 1.000000000000000000, 0.000000000000000000 ) ) ;
#15062=AXIS2_PLACEMENT_3D ( 'NONE', #5559, #16022, #106352 ) ;
#15063=ORIENTED_EDGE ( 'NONE', *, *, #30562, .F. ) ;
#15064=ORIENTED_EDGE ( 'NONE', *, *, #78435, .T. ) ;
#15065=ADVANCED_FACE ( 'NONE', ( #119764 ), #7738, .T. ) ;
#15066=CARTESIAN_POINT ( 'NONE',  ( 9.349999999999919709, 2.500000000000000000, 1.918653347947321564 ) ) ;
#15067=FACE_BOUND ( 'NONE', #47752, .T. ) ;
#15068=DIRECTION ( 'NONE',  ( -0.000000000000000000, 1.000000000000000000, -0.000000000000000000 ) ) ;
#15069=CARTESIAN_POINT ( 'NONE',  ( -4.999999999999986677, 12.50000000000000000, -2.276824562219559311E-15 ) ) ;
#15070=VECTOR ( 'NONE', #123134, 1000.000000000000000 ) ;
#15071=CIRCLE ( 'NONE', #10875, 0.06509327318403745899 ) ;
#15072=CARTESIAN_POINT ( 'NONE',  ( 2.699999999999946443, 2.500000000000000000, 0.3464101615137735735 ) ) ;
#15073=EDGE_LOOP ( 'NONE', ( #57311, #27207, #97407, #33798 ) ) ;
#15074=CONICAL_SURFACE ( 'NONE', #10877, 0.09999999999999982514, 0.003490658503988666988 ) ;
#15076=CIRCLE ( 'NONE', #6766, 0.1000000000000002554 ) ;
#15077=ORIENTED_EDGE ( 'NONE', *, *, #102182, .F. ) ;
#15078=CARTESIAN_POINT ( 'NONE',  ( 7.049999999999930544, 2.500000000000000000, -6.395190528383301931 ) ) ;
#15079=CARTESIAN_POINT ( 'NONE',  ( 5.649999999999932854, 2.500000000000000000, 2.411473670974873862 ) ) ;
#15080=DIRECTION ( 'NONE',  ( 0.000000000000000000, -0.9999939076577903929, 0.003490651415223739937 ) ) ;
#15081=CONICAL_SURFACE ( 'NONE', #8840, 0.1000000000000000472, 0.003490658503988666988 ) ;
#15082=DIRECTION ( 'NONE',  ( 0.000000000000000000, 0.000000000000000000, 1.000000000000000000 ) ) ;
#15083=ORIENTED_EDGE ( 'NONE', *, *, #74094, .F. ) ;
#15084=DIRECTION ( 'NONE',  ( 0.000000000000000000, 0.000000000000000000, 1.000000000000000000 ) ) ;
#15085=CARTESIAN_POINT ( 'NONE',  ( 4.349999999999937472, 2.500000000000000000, 6.741600689897071952 ) ) ;
#15086=AXIS2_PLACEMENT_3D ( 'NONE', #105309, #33993, #25431 ) ;
#15087=ORIENTED_EDGE ( 'NONE', *, *, #113141, .T. ) ;
#15088=DIRECTION ( 'NONE',  ( 0.000000000000000000, 1.000000000000000000, 0.000000000000000000 ) ) ;
#15089=VERTEX_POINT ( 'NONE', #129614 ) ;
#15090=FACE_BOUND ( 'NONE', #83099, .T. ) ;
#15091=CARTESIAN_POINT ( 'NONE',  ( 8.749999999999920064, 2.500000000000000000, 5.902370205355745192 ) ) ;
#15092=EDGE_CURVE ( 'NONE', #105669, #32860, #76711, .T. ) ;
#15093=ORIENTED_EDGE ( 'NONE', *, *, #16743, .F. ) ;
#15094=CARTESIAN_POINT ( 'NONE',  ( -14.54999999999998472, 2.500000000000000000, 2.065063509461101621 ) ) ;
#15095=DIRECTION ( 'NONE',  ( -0.000000000000000000, 1.000000000000000000, -0.000000000000000000 ) ) ;
#15096=ORIENTED_EDGE ( 'NONE', *, *, #61719, .T. ) ;
#15097=EDGE_LOOP ( 'NONE', ( #81038, #41334 ) ) ;
#15100=EDGE_CURVE ( 'NONE', #78428, #81254, #87249, .T. ) ;
#15101=ORIENTED_EDGE ( 'NONE', *, *, #107527, .T. ) ;
#15102=DIRECTION ( 'NONE',  ( 0.000000000000000000, 0.000000000000000000, 1.000000000000000000 ) ) ;
#15104=AXIS2_PLACEMENT_3D ( 'NONE', #41556, #98501, #110904 ) ;
#15105=DIRECTION ( 'NONE',  ( 0.000000000000000000, -0.9999939076577903929, 0.003490651415223739937 ) ) ;
#15106=CARTESIAN_POINT ( 'NONE',  ( -12.04999999999999716, 2.500000000000000000, -6.495190528383298911 ) ) ;
#15107=EDGE_CURVE ( 'NONE', #123328, #12341, #39932, .T. ) ;
#15108=VECTOR ( 'NONE', #64787, 1000.000000000000000 ) ;
#15109=EDGE_CURVE ( 'NONE', #21310, #79729, #21569, .T. ) ;
#15110=CARTESIAN_POINT ( 'NONE',  ( -8.950000000000009948, 2.500000000000000000, -6.841600689897072485 ) ) ;
#15111=CARTESIAN_POINT ( 'NONE',  ( -4.600000000000028955, 2.500000000000000000, -4.330127018922201643 ) ) ;
#15112=EDGE_CURVE ( 'NONE', #55936, #105517, #79836, .T. ) ;
#15113=ADVANCED_FACE ( 'NONE', ( #61511 ), #90282, .T. ) ;
#15114=AXIS2_PLACEMENT_3D ( 'NONE', #51760, #82519, #120497 ) ;
#15115=CONICAL_SURFACE ( 'NONE', #4648, 0.1000000000000002554, 0.003490658503988666988 ) ;
#15116=EDGE_LOOP ( 'NONE', ( #28966, #121107, #63819, #28717 ) ) ;
#15117=AXIS2_PLACEMENT_3D ( 'NONE', #43864, #121113, #32111 ) ;
#15118=ORIENTED_EDGE ( 'NONE', *, *, #99724, .F. ) ;
#15119=DIRECTION ( 'NONE',  ( 0.000000000000000000, 0.000000000000000000, 1.000000000000000000 ) ) ;
#15120=ADVANCED_FACE ( 'NONE', ( #71973 ), #122774, .T. ) ;
#15121=CARTESIAN_POINT ( 'NONE',  ( -12.49999999999999289, 12.50000000000000000, 3.637306695894644726 ) ) ;
#15122=DIRECTION ( 'NONE',  ( 0.000000000000000000, -0.000000000000000000, 1.000000000000000000 ) ) ;
#15123=AXIS2_PLACEMENT_3D ( 'NONE', #21281, #61215, #3579 ) ;
#15124=FACE_OUTER_BOUND ( 'NONE', #8430, .T. ) ;
#15126=EDGE_LOOP ( 'NONE', ( #24841, #568, #100651, #95291 ) ) ;
#15127=EDGE_LOOP ( 'NONE', ( #69130, #40975, #12201, #29535 ) ) ;
#15128=FACE_BOUND ( 'NONE', #96406, .T. ) ;
#15129=VERTEX_POINT ( 'NONE', #11082 ) ;
#15130=DIRECTION ( 'NONE',  ( -4.274815082592931898E-19, -0.9999939076577903929, -0.003490651415223739937 ) ) ;
#15132=EDGE_CURVE ( 'NONE', #53696, #80576, #116212, .T. ) ;
#15133=CIRCLE ( 'NONE', #65227, 0.09999999999999982514 ) ;
#15134=ORIENTED_EDGE ( 'NONE', *, *, #92242, .T. ) ;
#15135=DIRECTION ( 'NONE',  ( 0.000000000000000000, 0.000000000000000000, -1.000000000000000000 ) ) ;
#15136=LINE ( 'NONE', #54433, #3411 ) ;
#15137=CARTESIAN_POINT ( 'NONE',  ( 7.049999999999930544, 12.50000000000000000, -6.430097255199264339 ) ) ;
#15138=CARTESIAN_POINT ( 'NONE',  ( 0.3999999999999563904, 2.500000000000000000, 3.537306695894645081 ) ) ;
#15139=DIRECTION ( 'NONE',  ( 0.000000000000000000, 0.000000000000000000, 1.000000000000000000 ) ) ;
#15140=DIRECTION ( 'NONE',  ( -0.000000000000000000, -1.000000000000000000, -0.000000000000000000 ) ) ;
#15141=CARTESIAN_POINT ( 'NONE',  ( 4.149999999999939959, 2.500000000000000000, -6.495190528383302464 ) ) ;
#15142=CARTESIAN_POINT ( 'NONE',  ( 1.049999999999953637, 2.500000000000000000, 2.611473670974873151 ) ) ;
#15143=CARTESIAN_POINT ( 'NONE',  ( 8.149999999999920419, 12.50000000000000000, -2.511473670974877948 ) ) ;
#15144=CIRCLE ( 'NONE', #61446, 0.09999999999999982514 ) ;
#15145=ORIENTED_EDGE ( 'NONE', *, *, #21835, .T. ) ;
#15146=VERTEX_POINT ( 'NONE', #1278 ) ;
#15147=CARTESIAN_POINT ( 'NONE',  ( 7.099999999999926814, 2.500000000000000000, -0.7928203230275542301 ) ) ;
#15148=ORIENTED_EDGE ( 'NONE', *, *, #110622, .T. ) ;
#15149=CARTESIAN_POINT ( 'NONE',  ( 20.80940928220344688, 0.7000174339600965245, 4.161255421338325711 ) ) ;
#15150=ORIENTED_EDGE ( 'NONE', *, *, #76831, .T. ) ;
#15151=ORIENTED_EDGE ( 'NONE', *, *, #93511, .F. ) ;
#15152=ORIENTED_EDGE ( 'NONE', *, *, #12458, .T. ) ;
#15153=FACE_OUTER_BOUND ( 'NONE', #105076, .T. ) ;
#15154=AXIS2_PLACEMENT_3D ( 'NONE', #89297, #48742, #70949 ) ;
#15155=VECTOR ( 'NONE', #115245, 1000.000000000000000 ) ;
#15156=CARTESIAN_POINT ( 'NONE',  ( 14.79999999999989413, 2.500000000000000000, -0.3464101615137782364 ) ) ;
#15157=CARTESIAN_POINT ( 'NONE',  ( -3.750000000000025757, 2.500000000000000000, 1.372243186433545370 ) ) ;
#15158=CARTESIAN_POINT ( 'NONE',  ( 11.24999999999990941, 2.500000000000000000, 7.288010851410849256 ) ) ;
#15159=CARTESIAN_POINT ( 'NONE',  ( 1.899999999999951283, 12.50000000000000000, -0.3464101615137782364 ) ) ;
#15160=EDGE_LOOP ( 'NONE', ( #99157, #30438, #126273, #51123 ) ) ;
#15161=AXIS2_PLACEMENT_3D ( 'NONE', #124741, #15412, #85454 ) ;
#15163=DIRECTION ( 'NONE',  ( -0.000000000000000000, 1.000000000000000000, -0.000000000000000000 ) ) ;
#15164=EDGE_LOOP ( 'NONE', ( #42159, #97596, #5935, #80424 ) ) ;
#15165=CONICAL_SURFACE ( 'NONE', #59117, 0.1000000000000002554, 0.003490658503988666988 ) ;
#15166=VERTEX_POINT ( 'NONE', #101422 ) ;
#15167=AXIS2_PLACEMENT_3D ( 'NONE', #83968, #123895, #112806 ) ;
#15168=ADVANCED_FACE ( 'NONE', ( #51686 ), #47567, .T. ) ;
#15169=EDGE_LOOP ( 'NONE', ( #30768, #69915 ) ) ;
#15170=DIRECTION ( 'NONE',  ( 0.000000000000000000, 1.000000000000000000, 0.000000000000000000 ) ) ;
#15171=ORIENTED_EDGE ( 'NONE', *, *, #118530, .T. ) ;
#15172=ORIENTED_EDGE ( 'NONE', *, *, #19447, .F. ) ;
#15173=ORIENTED_EDGE ( 'NONE', *, *, #34342, .F. ) ;
#15174=CIRCLE ( 'NONE', #61172, 0.1000000000000002554 ) ;
#15175=DIRECTION ( 'NONE',  ( 0.000000000000000000, 0.000000000000000000, 1.000000000000000000 ) ) ;
#15176=AXIS2_PLACEMENT_3D ( 'NONE', #55693, #5930, #66154 ) ;
#15177=ADVANCED_FACE ( 'NONE', ( #113820 ), #28692, .T. ) ;
#15178=CARTESIAN_POINT ( 'NONE',  ( 6.849999999999929479, 2.500000000000000000, -1.818653347947326138 ) ) ;
#15179=CARTESIAN_POINT ( 'NONE',  ( 9.599999999999914380, 2.500000000000000000, 3.537306695894645081 ) ) ;
#15180=CARTESIAN_POINT ( 'NONE',  ( 9.599999999999914380, 12.50000000000000000, -3.637306695894650055 ) ) ;
#15181=CIRCLE ( 'NONE', #88338, 0.06509327318403741736 ) ;
#15182=DIRECTION ( 'NONE',  ( -0.000000000000000000, 1.000000000000000000, -0.000000000000000000 ) ) ;
#15183=AXIS2_PLACEMENT_3D ( 'NONE', #42267, #1673, #69279 ) ;
#15184=DIRECTION ( 'NONE',  ( 0.000000000000000000, 0.000000000000000000, 1.000000000000000000 ) ) ;
#15185=ORIENTED_EDGE ( 'NONE', *, *, #12195, .F. ) ;
#15186=AXIS2_PLACEMENT_3D ( 'NONE', #3230, #54257, #112545 ) ;
#15187=DIRECTION ( 'NONE',  ( 0.000000000000000000, 0.000000000000000000, 1.000000000000000000 ) ) ;
#15188=EDGE_LOOP ( 'NONE', ( #95930, #9057 ) ) ;
#15189=LINE ( 'NONE', #66239, #96540 ) ;
#15190=ORIENTED_EDGE ( 'NONE', *, *, #88462, .F. ) ;
#15191=DIRECTION ( 'NONE',  ( 0.000000000000000000, 0.000000000000000000, -1.000000000000000000 ) ) ;
#15192=VERTEX_POINT ( 'NONE', #115076 ) ;
#15193=ORIENTED_EDGE ( 'NONE', *, *, #103053, .F. ) ;
#15194=CARTESIAN_POINT ( 'NONE',  ( -8.749999999999971578, 12.50000000000000000, 6.495190528383297135 ) ) ;
#15195=CARTESIAN_POINT ( 'NONE',  ( -10.00000000000000533, 2.500000000000000000, -5.022947341949749678 ) ) ;
#15196=DIRECTION ( 'NONE',  ( 0.000000000000000000, 0.000000000000000000, 1.000000000000000000 ) ) ;
#15197=CARTESIAN_POINT ( 'NONE',  ( -1.850000000000033840, 12.50000000000000000, 1.818653347947321475 ) ) ;
#15198=VERTEX_POINT ( 'NONE', #24150 ) ;
#15199=DIRECTION ( 'NONE',  ( -0.000000000000000000, 1.000000000000000000, -0.000000000000000000 ) ) ;
#15200=CARTESIAN_POINT ( 'NONE',  ( 3.749999999999976907, 12.50000000000000000, 2.165063509461097713 ) ) ;
#15201=AXIS2_PLACEMENT_3D ( 'NONE', #20351, #120482, #60300 ) ;
#15202=AXIS2_PLACEMENT_3D ( 'NONE', #49062, #38601, #16334 ) ;
#15203=CARTESIAN_POINT ( 'NONE',  ( 0.7999999999999548583, 2.500000000000000000, 4.230127018922196669 ) ) ;
#15204=CARTESIAN_POINT ( 'NONE',  ( -1.850000000000033840, 12.50000000000000000, 6.841600689897072485 ) ) ;
#15205=CARTESIAN_POINT ( 'NONE',  ( -0.8500000000000382805, 2.500000000000000000, -1.572243186433550211 ) ) ;
#15206=ADVANCED_FACE ( 'NONE', ( #104625 ), #16135, .T. ) ;
#15207=EDGE_LOOP ( 'NONE', ( #71, #111091, #100800, #90692 ) ) ;
#15208=CIRCLE ( 'NONE', #8860, 0.06509327318403745899 ) ;
#15209=ORIENTED_EDGE ( 'NONE', *, *, #117889, .T. ) ;
#15210=AXIS2_PLACEMENT_3D ( 'NONE', #56843, #125592, #96775 ) ;
#15211=CIRCLE ( 'NONE', #84282, 0.06509327318403745899 ) ;
#15212=ORIENTED_EDGE ( 'NONE', *, *, #94242, .F. ) ;
#15213=CARTESIAN_POINT ( 'NONE',  ( -2.499999999999996003, 2.500000000000000000, -4.330127018922201643 ) ) ;
#15214=LINE ( 'NONE', #85900, #35589 ) ;
#15215=EDGE_CURVE ( 'NONE', #50751, #100973, #120716, .T. ) ;
#15216=AXIS2_PLACEMENT_3D ( 'NONE', #67332, #28749, #17614 ) ;
#15217=AXIS2_PLACEMENT_3D ( 'NONE', #26675, #66587, #16183 ) ;
#15218=CIRCLE ( 'NONE', #63265, 0.06509327318403745899 ) ;
#15220=ADVANCED_FACE ( 'NONE', ( #105286 ), #9612, .T. ) ;
#15222=CARTESIAN_POINT ( 'NONE',  ( -5.000000000000026645, 2.500000000000000000, -3.537306695894649966 ) ) ;
#15223=DIRECTION ( 'NONE',  ( 0.000000000000000000, 1.000000000000000000, 0.000000000000000000 ) ) ;
#15224=CARTESIAN_POINT ( 'NONE',  ( -3.100000000000028511, 12.50000000000000000, -4.676537180435977881 ) ) ;
#15225=EDGE_CURVE ( 'NONE', #40372, #127950, #76806, .T. ) ;
#15227=ORIENTED_EDGE ( 'NONE', *, *, #73936, .F. ) ;
#15228=CONICAL_SURFACE ( 'NONE', #69527, 0.09999999999999982514, 0.003490658503988666988 ) ;
#15229=LINE ( 'NONE', #47301, #48522 ) ;
#15230=DIRECTION ( 'NONE',  ( -4.274815082592931898E-19, -0.9999939076577903929, -0.003490651415223739937 ) ) ;
#15231=ADVANCED_FACE ( 'NONE', ( #3853 ), #57938, .T. ) ;
#15232=ORIENTED_EDGE ( 'NONE', *, *, #122870, .T. ) ;
#15233=ADVANCED_FACE ( 'NONE', ( #84985 ), #53817, .T. ) ;
#15234=DIRECTION ( 'NONE',  ( 0.000000000000000000, 1.000000000000000000, 0.000000000000000000 ) ) ;
#15235=LINE ( 'NONE', #112179, #94985 ) ;
#15236=CIRCLE ( 'NONE', #32006, 0.06509327318403745899 ) ;
#15237=ORIENTED_EDGE ( 'NONE', *, *, #99515, .F. ) ;
#15238=DIRECTION ( 'NONE',  ( 0.000000000000000000, 0.000000000000000000, -1.000000000000000000 ) ) ;
#15239=ORIENTED_EDGE ( 'NONE', *, *, #53878, .F. ) ;
#15240=DIRECTION ( 'NONE',  ( -0.000000000000000000, -1.000000000000000000, -0.000000000000000000 ) ) ;
#15241=CARTESIAN_POINT ( 'NONE',  ( -1.650000000000034772, 2.500000000000000000, 1.472243186433545459 ) ) ;
#15242=CARTESIAN_POINT ( 'NONE',  ( -4.350000000000027178, 2.500000000000000000, -6.941600689897077459 ) ) ;
#15243=AXIS2_PLACEMENT_3D ( 'NONE', #86560, #26370, #17142 ) ;
#15244=VERTEX_POINT ( 'NONE', #4473 ) ;
#15245=CONICAL_SURFACE ( 'NONE', #117647, 0.09999999999999999167, 0.003490658503988666988 ) ;
#15246=DIRECTION ( 'NONE',  ( 0.000000000000000000, 0.000000000000000000, -1.000000000000000000 ) ) ;
#15247=DIRECTION ( 'NONE',  ( -0.000000000000000000, 1.000000000000000000, -0.000000000000000000 ) ) ;
#15248=AXIS2_PLACEMENT_3D ( 'NONE', #17681, #26233, #106076 ) ;
#15249=VERTEX_POINT ( 'NONE', #43165 ) ;
#15250=VECTOR ( 'NONE', #83001, 1000.000000000000000 ) ;
#15251=DIRECTION ( 'NONE',  ( -4.274815082592931898E-19, -0.9999939076577903929, -0.003490651415223739937 ) ) ;
#15252=CONICAL_SURFACE ( 'NONE', #88433, 0.1000000000000002554, 0.003490658503988666988 ) ;
#15254=ORIENTED_EDGE ( 'NONE', *, *, #42005, .T. ) ;
#15255=DIRECTION ( 'NONE',  ( 0.000000000000000000, 0.000000000000000000, 1.000000000000000000 ) ) ;
#15256=DIRECTION ( 'NONE',  ( 0.000000000000000000, -0.9999939076577903929, 0.003490651415223739937 ) ) ;
#15257=VERTEX_POINT ( 'NONE', #35897 ) ;
#15258=DIRECTION ( 'NONE',  ( -0.000000000000000000, 1.000000000000000000, -0.000000000000000000 ) ) ;
#15259=CARTESIAN_POINT ( 'NONE',  ( -12.69999999999999396, 2.500000000000000000, 0.3464101615137776813 ) ) ;
#15260=AXIS2_PLACEMENT_3D ( 'NONE', #45717, #105920, #26713 ) ;
#15261=ORIENTED_EDGE ( 'NONE', *, *, #41673, .T. ) ;
#15262=ADVANCED_FACE ( 'NONE', ( #94817 ), #20373, .T. ) ;
#15263=FACE_OUTER_BOUND ( 'NONE', #108302, .T. ) ;
#15264=CARTESIAN_POINT ( 'NONE',  ( 1.049999999999953637, 2.500000000000000000, 2.411473670974873862 ) ) ;
#15265=CIRCLE ( 'NONE', #25664, 0.1000000000000000472 ) ;
#15266=CIRCLE ( 'NONE', #57152, 0.06509327318403745899 ) ;
#15267=AXIS2_PLACEMENT_3D ( 'NONE', #52854, #41121, #70551 ) ;
#15268=EDGE_CURVE ( 'NONE', #111073, #80386, #103362, .T. ) ;
#15269=CARTESIAN_POINT ( 'NONE',  ( -9.600000000000008527, 2.500000000000000000, -2.385244779468109755E-15 ) ) ;
#15270=CARTESIAN_POINT ( 'NONE',  ( -14.39999999999998614, 2.500000000000000000, 0.3464101615137758494 ) ) ;
#15271=EDGE_CURVE ( 'NONE', #57444, #51769, #93529, .T. ) ;
#15272=DIRECTION ( 'NONE',  ( 0.000000000000000000, 0.000000000000000000, -1.000000000000000000 ) ) ;
#15273=AXIS2_PLACEMENT_3D ( 'NONE', #100608, #98675, #69879 ) ;
#15274=CARTESIAN_POINT ( 'NONE',  ( -2.500000000000030642, 12.50000000000000000, -0.6928203230275541413 ) ) ;
#15275=EDGE_CURVE ( 'NONE', #120157, #43219, #62792, .T. ) ;
#15276=EDGE_CURVE ( 'NONE', #46240, #124608, #78877, .T. ) ;
#15277=ORIENTED_EDGE ( 'NONE', *, *, #85786, .F. ) ;
#15278=CIRCLE ( 'NONE', #105186, 0.1000000000000002554 ) ;
#15279=ORIENTED_EDGE ( 'NONE', *, *, #70280, .T. ) ;
#15280=ADVANCED_FACE ( 'NONE', ( #124924 ), #49631, .T. ) ;
#15281=ORIENTED_EDGE ( 'NONE', *, *, #23589, .T. ) ;
#15282=EDGE_LOOP ( 'NONE', ( #56569, #6183 ) ) ;
#15283=LINE ( 'NONE', #74877, #120630 ) ;
#15284=DIRECTION ( 'NONE',  ( 0.000000000000000000, -0.000000000000000000, 1.000000000000000000 ) ) ;
#15285=LINE ( 'NONE', #25770, #44741 ) ;
#15286=VERTEX_POINT ( 'NONE', #34632 ) ;
#15287=FACE_BOUND ( 'NONE', #95974, .T. ) ;
#15288=CARTESIAN_POINT ( 'NONE',  ( 11.64999999999990798, 2.500000000000000000, -1.372243186433550033 ) ) ;
#15289=FACE_OUTER_BOUND ( 'NONE', #97125, .T. ) ;
#15290=ADVANCED_FACE ( 'NONE', ( #125553 ), #13666, .T. ) ;
#15291=DIRECTION ( 'NONE',  ( 0.000000000000000000, -0.000000000000000000, 1.000000000000000000 ) ) ;
#15292=EDGE_CURVE ( 'NONE', #40372, #96407, #3226, .T. ) ;
#15293=DIRECTION ( 'NONE',  ( 0.000000000000000000, 0.000000000000000000, -1.000000000000000000 ) ) ;
#15294=CARTESIAN_POINT ( 'NONE',  ( -9.400000000000007461, 12.50000000000000000, -0.2813168883297409439 ) ) ;
#15295=DIRECTION ( 'NONE',  ( 0.000000000000000000, 1.000000000000000000, 0.000000000000000000 ) ) ;
#15296=CARTESIAN_POINT ( 'NONE',  ( -12.29999999999999538, 2.500000000000000000, -0.3464101615137741841 ) ) ;
#15297=DIRECTION ( 'NONE',  ( 0.000000000000000000, 0.000000000000000000, 1.000000000000000000 ) ) ;
#15298=CIRCLE ( 'NONE', #2799, 0.06509327318403745899 ) ;
#15299=DIRECTION ( 'NONE',  ( 0.000000000000000000, 1.000000000000000000, 0.000000000000000000 ) ) ;
#15300=CARTESIAN_POINT ( 'NONE',  ( 1.649999999999951950, 2.500000000000000000, -7.188010851410854052 ) ) ;
#15301=AXIS2_PLACEMENT_3D ( 'NONE', #126004, #38963, #118774 ) ;
#15302=ORIENTED_EDGE ( 'NONE', *, *, #34273, .T. ) ;
#15303=EDGE_LOOP ( 'NONE', ( #56884, #81256, #73255, #99373 ) ) ;
#15304=ORIENTED_EDGE ( 'NONE', *, *, #26978, .F. ) ;
#15305=ORIENTED_EDGE ( 'NONE', *, *, #27110, .F. ) ;
#15306=DIRECTION ( 'NONE',  ( 0.000000000000000000, 0.000000000000000000, 1.000000000000000000 ) ) ;
#15307=CONICAL_SURFACE ( 'NONE', #38326, 0.09999999999999982514, 0.003490658503988666988 ) ;
#15308=EDGE_LOOP ( 'NONE', ( #54296, #93829, #36769, #124835 ) ) ;
#15309=CIRCLE ( 'NONE', #121833, 0.06509327318403745899 ) ;
#15310=DIRECTION ( 'NONE',  ( 0.000000000000000000, 0.000000000000000000, -1.000000000000000000 ) ) ;
#15311=EDGE_LOOP ( 'NONE', ( #97665, #24979, #41018, #117569 ) ) ;
#15312=EDGE_CURVE ( 'NONE', #69366, #60185, #112315, .T. ) ;
#15313=EDGE_LOOP ( 'NONE', ( #85251, #17848, #51457, #1203 ) ) ;
#15314=FACE_OUTER_BOUND ( 'NONE', #78462, .T. ) ;
#15315=CIRCLE ( 'NONE', #11213, 0.06509327318403741736 ) ;
#15316=CIRCLE ( 'NONE', #38334, 0.09999999999999982514 ) ;
#15317=AXIS2_PLACEMENT_3D ( 'NONE', #61835, #32391, #33649 ) ;
#15318=CARTESIAN_POINT ( 'NONE',  ( 7.099999999999926814, 2.500000000000000000, -0.6928203230275541413 ) ) ;
#15319=DIRECTION ( 'NONE',  ( 0.000000000000000000, 0.000000000000000000, -1.000000000000000000 ) ) ;
#15320=DIRECTION ( 'NONE',  ( -0.000000000000000000, 1.000000000000000000, -0.000000000000000000 ) ) ;
#15321=CIRCLE ( 'NONE', #82247, 0.06509327318403745899 ) ;
#15322=DIRECTION ( 'NONE',  ( 0.000000000000000000, -0.000000000000000000, 1.000000000000000000 ) ) ;
#15323=CONICAL_SURFACE ( 'NONE', #57099, 0.1000000000000002554, 0.003490658503988666988 ) ;
#15324=ORIENTED_EDGE ( 'NONE', *, *, #121060, .F. ) ;
#15325=ORIENTED_EDGE ( 'NONE', *, *, #89636, .F. ) ;
#15326=ORIENTED_EDGE ( 'NONE', *, *, #41302, .T. ) ;
#15327=DIRECTION ( 'NONE',  ( 0.000000000000000000, 1.000000000000000000, 0.000000000000000000 ) ) ;
#15328=VERTEX_POINT ( 'NONE', #74534 ) ;
#15329=CARTESIAN_POINT ( 'NONE',  ( 7.499999999999925393, 2.500000000000000000, -3.637306695894650055 ) ) ;
#15330=ORIENTED_EDGE ( 'NONE', *, *, #3427, .T. ) ;
#15331=ORIENTED_EDGE ( 'NONE', *, *, #60760, .T. ) ;
#15332=CIRCLE ( 'NONE', #88501, 0.06509327318403745899 ) ;
#15333=DIRECTION ( 'NONE',  ( 0.000000000000000000, -0.9999939076577903929, 0.003490651415223739937 ) ) ;
#15334=EDGE_CURVE ( 'NONE', #99444, #80386, #72608, .T. ) ;
#15335=CARTESIAN_POINT ( 'NONE',  ( -4.200000000000025935, 2.500000000000000000, 4.430127018922196847 ) ) ;
#15336=DIRECTION ( 'NONE',  ( 0.000000000000000000, 0.000000000000000000, 1.000000000000000000 ) ) ;
#15337=PLANE ( 'NONE',  #100624 ) ;
#15338=PLANE ( 'NONE',  #50370 ) ;
#15339=CONICAL_SURFACE ( 'NONE', #111500, 0.1000000000000002554, 0.003490658503988666988 ) ;
#15340=EDGE_LOOP ( 'NONE', ( #23330, #24525, #121737, #113567 ) ) ;
#15341=CARTESIAN_POINT ( 'NONE',  ( -1.450000000000036371, 2.500000000000000000, 6.741600689897071952 ) ) ;
#15342=AXIS2_PLACEMENT_3D ( 'NONE', #101595, #49938, #89831 ) ;
#15343=AXIS2_PLACEMENT_3D ( 'NONE', #87380, #27821, #38977 ) ;
#15344=VERTEX_POINT ( 'NONE', #18827 ) ;
#15345=FACE_OUTER_BOUND ( 'NONE', #2121, .T. ) ;
#15346=EDGE_LOOP ( 'NONE', ( #60463, #50607, #74559, #69992 ) ) ;
#15348=DIRECTION ( 'NONE',  ( 0.000000000000000000, 1.000000000000000000, 0.000000000000000000 ) ) ;
#15349=CARTESIAN_POINT ( 'NONE',  ( -3.350000000000028955, 2.500000000000000000, 7.288010851410849256 ) ) ;
#15350=LINE ( 'NONE', #62557, #58483 ) ;
#15351=ORIENTED_EDGE ( 'NONE', *, *, #105276, .T. ) ;
#15352=CIRCLE ( 'NONE', #84328, 0.09999999999999982514 ) ;
#15353=AXIS2_PLACEMENT_3D ( 'NONE', #8877, #96609, #9550 ) ;
#15354=CARTESIAN_POINT ( 'NONE',  ( -4.400000000000025224, 2.500000000000000000, -0.3464101615137783474 ) ) ;
#15355=VECTOR ( 'NONE', #79020, 1000.000000000000000 ) ;
#15356=DIRECTION ( 'NONE',  ( 0.000000000000000000, 0.000000000000000000, -1.000000000000000000 ) ) ;
#15357=ORIENTED_EDGE ( 'NONE', *, *, #34308, .F. ) ;
#15358=VERTEX_POINT ( 'NONE', #58762 ) ;
#15359=VERTEX_POINT ( 'NONE', #39149 ) ;
#15360=CARTESIAN_POINT ( 'NONE',  ( 9.599999999999914380, 2.500000000000000000, -4.922947341949753586 ) ) ;
#15361=DIRECTION ( 'NONE',  ( 0.000000000000000000, 0.000000000000000000, 1.000000000000000000 ) ) ;
#15363=AXIS2_PLACEMENT_3D ( 'NONE', #105801, #44956, #84865 ) ;
#15364=FACE_OUTER_BOUND ( 'NONE', #107830, .T. ) ;
#15365=DIRECTION ( 'NONE',  ( 0.000000000000000000, 1.000000000000000000, 0.000000000000000000 ) ) ;
#15366=CIRCLE ( 'NONE', #4908, 0.1000000000000002554 ) ;
#15367=CIRCLE ( 'NONE', #52960, 0.1000000000000002554 ) ;
#15368=AXIS2_PLACEMENT_3D ( 'NONE', #73768, #96002, #115623 ) ;
#15369=DIRECTION ( 'NONE',  ( 0.000000000000000000, 0.000000000000000000, 1.000000000000000000 ) ) ;
#15370=AXIS2_PLACEMENT_3D ( 'NONE', #58626, #39647, #120115 ) ;
#15371=ORIENTED_EDGE ( 'NONE', *, *, #106319, .T. ) ;
#15372=AXIS2_PLACEMENT_3D ( 'NONE', #3535, #76148, #26412 ) ;
#15373=CARTESIAN_POINT ( 'NONE',  ( -12.49999999999999289, 2.500000000000000000, -5.022947341949751454 ) ) ;
#15374=ADVANCED_FACE ( 'NONE', ( #48296 ), #126980, .T. ) ;
#15375=ORIENTED_EDGE ( 'NONE', *, *, #125426, .F. ) ;
#15376=EDGE_CURVE ( 'NONE', #48300, #107800, #14088, .T. ) ;
#15377=DIRECTION ( 'NONE',  ( 0.000000000000000000, -0.9999939076577903929, 0.003490651415223739937 ) ) ;
#15378=DIRECTION ( 'NONE',  ( 0.000000000000000000, 1.000000000000000000, 0.000000000000000000 ) ) ;
#15379=DIRECTION ( 'NONE',  ( 0.000000000000000000, 1.000000000000000000, 0.000000000000000000 ) ) ;
#15380=EDGE_CURVE ( 'NONE', #96527, #117477, #3356, .T. ) ;
#15381=ORIENTED_EDGE ( 'NONE', *, *, #70847, .T. ) ;
#15382=DIRECTION ( 'NONE',  ( 0.000000000000000000, 1.000000000000000000, 0.000000000000000000 ) ) ;
#15383=DIRECTION ( 'NONE',  ( 0.000000000000000000, 0.000000000000000000, -1.000000000000000000 ) ) ;
#15384=EDGE_CURVE ( 'NONE', #119064, #124197, #91376, .T. ) ;
#15385=EDGE_CURVE ( 'NONE', #84066, #41827, #26723, .T. ) ;
#15386=CONICAL_SURFACE ( 'NONE', #7068, 0.09999999999999982514, 0.003490658503988666988 ) ;
#15387=CIRCLE ( 'NONE', #27930, 0.06509327318403745899 ) ;
#15388=ADVANCED_FACE ( 'NONE', ( #46348 ), #97439, .T. ) ;
#15389=EDGE_CURVE ( 'NONE', #69025, #56716, #41033, .T. ) ;
#15390=EDGE_LOOP ( 'NONE', ( #38042, #68883, #117598, #127860 ) ) ;
#15391=DIRECTION ( 'NONE',  ( 0.000000000000000000, 0.000000000000000000, 1.000000000000000000 ) ) ;
#15392=AXIS2_PLACEMENT_3D ( 'NONE', #13962, #5432, #114109 ) ;
#15393=AXIS2_PLACEMENT_3D ( 'NONE', #124211, #70758, #114378 ) ;
#15394=ORIENTED_EDGE ( 'NONE', *, *, #42028, .F. ) ;
#15395=ORIENTED_EDGE ( 'NONE', *, *, #86931, .F. ) ;
#15396=DIRECTION ( 'NONE',  ( -0.000000000000000000, 1.000000000000000000, -0.000000000000000000 ) ) ;
#15397=CIRCLE ( 'NONE', #50943, 0.06509327318403745899 ) ;
#15398=VECTOR ( 'NONE', #10687, 1000.000000000000000 ) ;
#15399=EDGE_CURVE ( 'NONE', #2985, #107746, #7706, .T. ) ;
#15400=ORIENTED_EDGE ( 'NONE', *, *, #83395, .T. ) ;
#15401=CARTESIAN_POINT ( 'NONE',  ( 17.29982614915083161, 2.489966891809608285, -2.989943721782188479 ) ) ;
#15403=CARTESIAN_POINT ( 'NONE',  ( 4.799999999999937650, 2.500000000000000000, -0.3464101615137782364 ) ) ;
#15404=AXIS2_PLACEMENT_3D ( 'NONE', #19601, #57599, #48410 ) ;
#15405=ORIENTED_EDGE ( 'NONE', *, *, #12849, .T. ) ;
#15406=AXIS2_PLACEMENT_3D ( 'NONE', #46566, #75379, #14522 ) ;
#15407=CIRCLE ( 'NONE', #67650, 0.09999999999999982514 ) ;
#15408=FACE_BOUND ( 'NONE', #123628, .T. ) ;
#15409=DIRECTION ( 'NONE',  ( 0.000000000000000000, 0.000000000000000000, 1.000000000000000000 ) ) ;
#15410=EDGE_LOOP ( 'NONE', ( #88311, #103083, #97618, #129414 ) ) ;
#15411=AXIS2_PLACEMENT_3D ( 'NONE', #41314, #72057, #111978 ) ;
#15412=DIRECTION ( 'NONE',  ( 0.000000000000000000, 1.000000000000000000, 0.000000000000000000 ) ) ;
#15413=CARTESIAN_POINT ( 'NONE',  ( 1.049999999999954969, 12.50000000000000000, -6.906693963081115051 ) ) ;
#15414=ORIENTED_EDGE ( 'NONE', *, *, #45858, .F. ) ;
#15415=ORIENTED_EDGE ( 'NONE', *, *, #101197, .F. ) ;
#15416=ORIENTED_EDGE ( 'NONE', *, *, #118594, .F. ) ;
#15417=DIRECTION ( 'NONE',  ( 0.000000000000000000, 0.000000000000000000, 1.000000000000000000 ) ) ;
#15418=CARTESIAN_POINT ( 'NONE',  ( -11.24999999999996270, 2.500000000000000000, 2.165063509461097713 ) ) ;
#15419=CARTESIAN_POINT ( 'NONE',  ( 0.5999999999999612310, 2.500000000000000000, -0.2464101615137760659 ) ) ;
#15420=ADVANCED_FACE ( 'NONE', ( #108493 ), #93250, .T. ) ;
#15421=FACE_BOUND ( 'NONE', #73247, .T. ) ;
#15422=EDGE_LOOP ( 'NONE', ( #50693, #82002 ) ) ;
#15424=DIRECTION ( 'NONE',  ( -4.274815082592931898E-19, -0.9999939076577903929, -0.003490651415223739937 ) ) ;
#15425=DIRECTION ( 'NONE',  ( 0.000000000000000000, 0.000000000000000000, 1.000000000000000000 ) ) ;
#15426=CONICAL_SURFACE ( 'NONE', #65617, 0.1000000000000002554, 0.003490658503988666988 ) ;
#15428=CARTESIAN_POINT ( 'NONE',  ( 4.549999999999939426, 12.50000000000000000, -2.165063509461101710 ) ) ;
#15429=FACE_OUTER_BOUND ( 'NONE', #121425, .T. ) ;
#15430=ADVANCED_FACE ( 'NONE', ( #47661 ), #16860, .T. ) ;
#15431=CARTESIAN_POINT ( 'NONE',  ( -11.89999999999999680, 2.500000000000000000, 0.3464101615137776813 ) ) ;
#15432=DIRECTION ( 'NONE',  ( -0.000000000000000000, 1.000000000000000000, -0.000000000000000000 ) ) ;
#15433=CONICAL_SURFACE ( 'NONE', #54870, 0.1000000000000002554, 0.003490658503988666988 ) ;
#15434=ADVANCED_FACE ( 'NONE', ( #86919 ), #49440, .T. ) ;
#15436=ADVANCED_FACE ( 'NONE', ( #28665 ), #30569, .T. ) ;
#15437=ORIENTED_EDGE ( 'NONE', *, *, #28941, .F. ) ;
#15438=VERTEX_POINT ( 'NONE', #38500 ) ;
#15439=ORIENTED_EDGE ( 'NONE', *, *, #68784, .F. ) ;
#15440=VERTEX_POINT ( 'NONE', #107207 ) ;
#15441=ORIENTED_EDGE ( 'NONE', *, *, #77361, .T. ) ;
#15443=CARTESIAN_POINT ( 'NONE',  ( 15.79999999999989058, 2.500000000000000000, -2.385244779468109755E-15 ) ) ;
#15444=ORIENTED_EDGE ( 'NONE', *, *, #100439, .F. ) ;
#15445=EDGE_CURVE ( 'NONE', #20339, #37854, #86975, .T. ) ;
#15446=FACE_BOUND ( 'NONE', #123537, .T. ) ;
#15447=AXIS2_PLACEMENT_3D ( 'NONE', #85479, #56006, #6890 ) ;
#15448=DIRECTION ( 'NONE',  ( 0.000000000000000000, 0.000000000000000000, 1.000000000000000000 ) ) ;
#15449=ADVANCED_FACE ( 'NONE', ( #96100 ), #91188, .T. ) ;
#15450=AXIS2_PLACEMENT_3D ( 'NONE', #123362, #84072, #73605 ) ;
#15451=ADVANCED_FACE ( 'NONE', ( #58126 ), #98034, .T. ) ;
#15452=CIRCLE ( 'NONE', #57236, 0.09999999999999982514 ) ;
#15453=EDGE_CURVE ( 'NONE', #40839, #83875, #126699, .T. ) ;
#15455=ORIENTED_EDGE ( 'NONE', *, *, #54293, .F. ) ;
#15456=DIRECTION ( 'NONE',  ( -0.000000000000000000, 1.000000000000000000, -0.000000000000000000 ) ) ;
#15459=ORIENTED_EDGE ( 'NONE', *, *, #16281, .F. ) ;
#15460=DIRECTION ( 'NONE',  ( -0.000000000000000000, 1.000000000000000000, -0.000000000000000000 ) ) ;
#15461=EDGE_CURVE ( 'NONE', #11368, #88940, #121528, .T. ) ;
#15462=ORIENTED_EDGE ( 'NONE', *, *, #58466, .F. ) ;
#15463=AXIS2_PLACEMENT_3D ( 'NONE', #76131, #34292, #116050 ) ;
#15464=CONICAL_SURFACE ( 'NONE', #13316, 0.1000000000000000056, 0.003490658503988666988 ) ;
#15465=AXIS2_PLACEMENT_3D ( 'NONE', #51431, #80234, #31776 ) ;
#15466=ORIENTED_EDGE ( 'NONE', *, *, #36312, .F. ) ;
#15468=LINE ( 'NONE', #55412, #59242 ) ;
#15469=DIRECTION ( 'NONE',  ( 0.000000000000000000, 1.000000000000000000, 0.000000000000000000 ) ) ;
#15470=CARTESIAN_POINT ( 'NONE',  ( -6.650000000000014566, 12.50000000000000000, 2.165063509461097713 ) ) ;
#15471=AXIS2_PLACEMENT_3D ( 'NONE', #97730, #89841, #8056 ) ;
#15472=ORIENTED_EDGE ( 'NONE', *, *, #69313, .T. ) ;
#15473=CARTESIAN_POINT ( 'NONE',  ( 13.80955901302282030, 2.500000000000000444, -7.955427456728518365 ) ) ;
#15474=CIRCLE ( 'NONE', #105375, 0.1000000000000002554 ) ;
#15475=CARTESIAN_POINT ( 'NONE',  ( 1.449999999999952660, 2.500000000000000000, -6.741600689897078169 ) ) ;
#15476=CARTESIAN_POINT ( 'NONE',  ( 6.849999999999929479, 12.50000000000000000, 6.148780366869520009 ) ) ;
#15478=CARTESIAN_POINT ( 'NONE',  ( 8.549999999999924327, 2.500000000000000000, 1.818653347947321475 ) ) ;
#15479=DIRECTION ( 'NONE',  ( -0.000000000000000000, -1.000000000000000000, -0.000000000000000000 ) ) ;
#15481=CARTESIAN_POINT ( 'NONE',  ( -0.2000000000000399791, 2.500000000000000000, -4.676537180435977881 ) ) ;
#15482=VERTEX_POINT ( 'NONE', #31244 ) ;
#15483=ORIENTED_EDGE ( 'NONE', *, *, #108359, .F. ) ;
#15484=DIRECTION ( 'NONE',  ( 0.000000000000000000, 0.000000000000000000, 1.000000000000000000 ) ) ;
#15485=CARTESIAN_POINT ( 'NONE',  ( -6.250000000000021316, 2.500000000000000000, -5.802370205355749988 ) ) ;
#15486=AXIS2_PLACEMENT_3D ( 'NONE', #122288, #33892, #32640 ) ;
#15487=CONICAL_SURFACE ( 'NONE', #2991, 0.09999999999999982514, 0.003490658503988666988 ) ;
#15488=DIRECTION ( 'NONE',  ( 0.000000000000000000, 0.000000000000000000, 1.000000000000000000 ) ) ;
#15489=AXIS2_PLACEMENT_3D ( 'NONE', #58160, #98060, #41749 ) ;
#15490=DIRECTION ( 'NONE',  ( -0.000000000000000000, -1.000000000000000000, -0.000000000000000000 ) ) ;
#15491=CARTESIAN_POINT ( 'NONE',  ( -4.150000000000025224, 2.500000000000000000, 7.288010851410849256 ) ) ;
#15493=ORIENTED_EDGE ( 'NONE', *, *, #55022, .T. ) ;
#15495=CONICAL_SURFACE ( 'NONE', #122136, 0.1000000000000002554, 0.003490658503988666988 ) ;
#15496=EDGE_CURVE ( 'NONE', #23794, #82143, #89506, .T. ) ;
#15497=VECTOR ( 'NONE', #110228, 1000.000000000000000 ) ;
#15498=CARTESIAN_POINT ( 'NONE',  ( -11.84999999999999609, 12.50000000000000000, 1.883746621131358934 ) ) ;
#15499=DIRECTION ( 'NONE',  ( -0.000000000000000000, -1.000000000000000000, -0.000000000000000000 ) ) ;
#15500=ORIENTED_EDGE ( 'NONE', *, *, #110002, .F. ) ;
#15501=ORIENTED_EDGE ( 'NONE', *, *, #105579, .F. ) ;
#15502=DIRECTION ( 'NONE',  ( 0.000000000000000000, 0.000000000000000000, -1.000000000000000000 ) ) ;
#15503=VERTEX_POINT ( 'NONE', #19469 ) ;
#15504=DIRECTION ( 'NONE',  ( 0.000000000000000000, 1.000000000000000000, 0.000000000000000000 ) ) ;
#15505=AXIS2_PLACEMENT_3D ( 'NONE', #109088, #107161, #118277 ) ;
#15506=AXIS2_PLACEMENT_3D ( 'NONE', #98111, #89593, #87003 ) ;
#15507=CARTESIAN_POINT ( 'NONE',  ( 6.649999999999930189, 2.500000000000000000, 7.188010851410848723 ) ) ;
#15508=VERTEX_POINT ( 'NONE', #120268 ) ;
#15509=DIRECTION ( 'NONE',  ( -0.000000000000000000, 1.000000000000000000, -0.000000000000000000 ) ) ;
#15510=DIRECTION ( 'NONE',  ( 0.000000000000000000, 0.000000000000000000, -1.000000000000000000 ) ) ;
#15511=DIRECTION ( 'NONE',  ( 0.000000000000000000, 0.000000000000000000, 1.000000000000000000 ) ) ;
#15512=AXIS2_PLACEMENT_3D ( 'NONE', #3793, #84927, #34566 ) ;
#15513=EDGE_CURVE ( 'NONE', #90471, #55194, #38992, .T. ) ;
#15514=DIRECTION ( 'NONE',  ( 0.000000000000000000, 1.000000000000000000, 0.000000000000000000 ) ) ;
#15515=EDGE_LOOP ( 'NONE', ( #14678, #21355 ) ) ;
#15516=CARTESIAN_POINT ( 'NONE',  ( 5.599999999999934808, 2.500000000000000000, -3.883716857408426648 ) ) ;
#15517=FACE_OUTER_BOUND ( 'NONE', #37686, .T. ) ;
#15518=ORIENTED_EDGE ( 'NONE', *, *, #45440, .T. ) ;
#15519=ORIENTED_EDGE ( 'NONE', *, *, #15550, .F. ) ;
#15521=CARTESIAN_POINT ( 'NONE',  ( -10.80000000000000071, 12.50000000000000000, 4.330127018922196314 ) ) ;
#15522=CARTESIAN_POINT ( 'NONE',  ( 0.6499999999999561684, 12.50000000000000000, -2.511473670974877948 ) ) ;
#15523=DIRECTION ( 'NONE',  ( 0.000000000000000000, 1.000000000000000000, 0.000000000000000000 ) ) ;
#15524=AXIS2_PLACEMENT_3D ( 'NONE', #47586, #37124, #86850 ) ;
#15525=CARTESIAN_POINT ( 'NONE',  ( 1.049999999999954525, 12.50000000000000000, 1.753560074763284016 ) ) ;
#15526=DIRECTION ( 'NONE',  ( -0.000000000000000000, 1.000000000000000000, -0.000000000000000000 ) ) ;
#15527=DIRECTION ( 'NONE',  ( -4.274815082592931898E-19, -0.9999939076577903929, -0.003490651415223739937 ) ) ;
#15528=DIRECTION ( 'NONE',  ( -0.000000000000000000, -1.000000000000000000, -0.000000000000000000 ) ) ;
#15529=CARTESIAN_POINT ( 'NONE',  ( -11.69999999999999574, 2.500000000000000000, 4.430127018922196847 ) ) ;
#15530=DIRECTION ( 'NONE',  ( 0.000000000000000000, 1.000000000000000000, 0.000000000000000000 ) ) ;
#15531=CARTESIAN_POINT ( 'NONE',  ( -4.400000000000025224, 12.50000000000000000, 0.3464101615137735735 ) ) ;
#15532=VECTOR ( 'NONE', #80995, 1000.000000000000000 ) ;
#15533=EDGE_LOOP ( 'NONE', ( #126270, #14600, #52581, #124186 ) ) ;
#15534=CIRCLE ( 'NONE', #113848, 0.1000000000000002554 ) ;
#15535=EDGE_CURVE ( 'NONE', #110459, #35601, #118963, .T. ) ;
#15536=VERTEX_POINT ( 'NONE', #30608 ) ;
#15537=ORIENTED_EDGE ( 'NONE', *, *, #82821, .F. ) ;
#15538=CARTESIAN_POINT ( 'NONE',  ( 10.64999999999991331, 2.500000000000000000, -2.411473670974877859 ) ) ;
#15539=CARTESIAN_POINT ( 'NONE',  ( -3.100000000000028955, 2.500000000000000000, 4.083716857408421497 ) ) ;
#15540=ADVANCED_FACE ( 'NONE', ( #10912 ), #26444, .T. ) ;
#15541=VERTEX_POINT ( 'NONE', #111723 ) ;
#15542=CARTESIAN_POINT ( 'NONE',  ( -11.05000000000000249, 12.50000000000000000, -6.083687093685485436 ) ) ;
#15543=AXIS2_PLACEMENT_3D ( 'NONE', #27164, #116180, #86062 ) ;
#15544=LINE ( 'NONE', #22825, #122326 ) ;
#15545=DIRECTION ( 'NONE',  ( -0.000000000000000000, -0.000000000000000000, -1.000000000000000000 ) ) ;
#15547=EDGE_CURVE ( 'NONE', #124884, #87296, #112128, .T. ) ;
#15548=EDGE_CURVE ( 'NONE', #35541, #14887, #124642, .T. ) ;
#15549=ADVANCED_FACE ( 'NONE', ( #40431 ), #61341, .T. ) ;
#15550=EDGE_CURVE ( 'NONE', #63288, #101710, #64000, .T. ) ;
#15551=FACE_OUTER_BOUND ( 'NONE', #52146, .T. ) ;
#15552=ORIENTED_EDGE ( 'NONE', *, *, #34939, .F. ) ;
#15553=AXIS2_PLACEMENT_3D ( 'NONE', #43947, #44584, #15084 ) ;
#15554=CONICAL_SURFACE ( 'NONE', #107609, 0.1000000000000002554, 0.003490658503988666988 ) ;
#15555=ORIENTED_EDGE ( 'NONE', *, *, #125216, .F. ) ;
#15556=ORIENTED_EDGE ( 'NONE', *, *, #73947, .T. ) ;
#15558=DIRECTION ( 'NONE',  ( 0.000000000000000000, 0.000000000000000000, -1.000000000000000000 ) ) ;
#15559=AXIS2_PLACEMENT_3D ( 'NONE', #50556, #102874, #21101 ) ;
#15560=EDGE_CURVE ( 'NONE', #110183, #128448, #68189, .T. ) ;
#15561=DIRECTION ( 'NONE',  ( 0.000000000000000000, 1.000000000000000000, 0.000000000000000000 ) ) ;
#15563=AXIS2_PLACEMENT_3D ( 'NONE', #70995, #30444, #31089 ) ;
#15564=ADVANCED_FACE ( 'NONE', ( #92071 ), #39785, .T. ) ;
#15565=FACE_OUTER_BOUND ( 'NONE', #103951, .T. ) ;
#15566=EDGE_CURVE ( 'NONE', #108298, #121302, #128870, .T. ) ;
#15567=ORIENTED_EDGE ( 'NONE', *, *, #58729, .T. ) ;
#15568=LINE ( 'NONE', #95438, #41847 ) ;
#15569=ORIENTED_EDGE ( 'NONE', *, *, #116488, .T. ) ;
#15570=CARTESIAN_POINT ( 'NONE',  ( 6.249999999999967137, 2.500000000000000000, 6.495190528383297135 ) ) ;
#15571=CARTESIAN_POINT ( 'NONE',  ( 8.949999999999915801, 2.500000000000000000, 6.741600689897071952 ) ) ;
#15572=DIRECTION ( 'NONE',  ( -4.274815082592931898E-19, -0.9999939076577903929, -0.003490651415223739937 ) ) ;
#15573=CARTESIAN_POINT ( 'NONE',  ( 15.24415751722998635, -2.474878586408709058, 4.460068884076466844 ) ) ;
#15574=ORIENTED_EDGE ( 'NONE', *, *, #53512, .F. ) ;
#15575=VECTOR ( 'NONE', #33424, 1000.000000000000000 ) ;
#15576=VERTEX_POINT ( 'NONE', #60702 ) ;
#15577=EDGE_LOOP ( 'NONE', ( #90002, #79765, #115077, #58619 ) ) ;
#15578=LINE ( 'NONE', #55529, #77436 ) ;
#15579=DIRECTION ( 'NONE',  ( 0.000000000000000000, 1.000000000000000000, 0.000000000000000000 ) ) ;
#15580=AXIS2_PLACEMENT_3D ( 'NONE', #65750, #84099, #25182 ) ;
#15581=CONICAL_SURFACE ( 'NONE', #19804, 0.1000000000000002554, 0.003490658503988666988 ) ;
#15582=DIRECTION ( 'NONE',  ( 0.000000000000000000, 1.000000000000000000, 0.000000000000000000 ) ) ;
#15583=FACE_BOUND ( 'NONE', #6587, .T. ) ;
#15584=FACE_OUTER_BOUND ( 'NONE', #111287, .T. ) ;
#15585=DIRECTION ( 'NONE',  ( -0.000000000000000000, -1.000000000000000000, -0.000000000000000000 ) ) ;
#15586=CARTESIAN_POINT ( 'NONE',  ( -0.4000000000000331624, 2.500000000000000000, -0.5928203230275518321 ) ) ;
#15587=DIRECTION ( 'NONE',  ( -0.000000000000000000, -1.000000000000000000, -0.000000000000000000 ) ) ;
#15588=AXIS2_PLACEMENT_3D ( 'NONE', #20191, #81054, #79124 ) ;
#15589=CIRCLE ( 'NONE', #117997, 0.09999999999999999167 ) ;
#15590=CIRCLE ( 'NONE', #63644, 0.09999999999999982514 ) ;
#15592=CONICAL_SURFACE ( 'NONE', #124566, 0.1000000000000002554, 0.003490658503988666988 ) ;
#15593=CARTESIAN_POINT ( 'NONE',  ( -5.450000000000023270, 12.50000000000000000, -6.495190528383302464 ) ) ;
#15594=CARTESIAN_POINT ( 'NONE',  ( 14.14999999999989733, 12.50000000000000000, 1.407149913249508000 ) ) ;
#15595=AXIS2_PLACEMENT_3D ( 'NONE', #82458, #22247, #41886 ) ;
#15596=CARTESIAN_POINT ( 'NONE',  ( -2.900000000000030109, 2.500000000000000000, -3.737306695894649700 ) ) ;
#15597=ORIENTED_EDGE ( 'NONE', *, *, #10115, .T. ) ;
#15598=VERTEX_POINT ( 'NONE', #41077 ) ;
#15599=ORIENTED_EDGE ( 'NONE', *, *, #84487, .T. ) ;
#15600=ORIENTED_EDGE ( 'NONE', *, *, #71510, .F. ) ;
#15601=CIRCLE ( 'NONE', #28140, 0.09999999999999982514 ) ;
#15602=CARTESIAN_POINT ( 'NONE',  ( 1.649999999999951950, 2.500000000000000000, -7.088010851410853519 ) ) ;
#15603=EDGE_CURVE ( 'NONE', #84188, #62406, #41712, .T. ) ;
#15604=FACE_BOUND ( 'NONE', #95795, .T. ) ;
#15605=PLANE ( 'NONE',  #22298 ) ;
#15606=EDGE_CURVE ( 'NONE', #16422, #128537, #5487, .T. ) ;
#15607=EDGE_CURVE ( 'NONE', #11040, #126889, #59911, .T. ) ;
#15608=ORIENTED_EDGE ( 'NONE', *, *, #31755, .F. ) ;
#15609=CARTESIAN_POINT ( 'NONE',  ( 35.04009662963678551, 1.562391656599548373, 4.793251516053341099 ) ) ;
#15610=DIRECTION ( 'NONE',  ( 0.000000000000000000, 1.000000000000000000, 0.000000000000000000 ) ) ;
#15611=AXIS2_PLACEMENT_3D ( 'NONE', #123872, #54494, #115995 ) ;
#15612=ORIENTED_EDGE ( 'NONE', *, *, #46582, .T. ) ;
#15613=DIRECTION ( 'NONE',  ( -0.000000000000000000, 1.000000000000000000, -0.000000000000000000 ) ) ;
#15614=DIRECTION ( 'NONE',  ( -0.000000000000000000, 1.000000000000000000, -0.000000000000000000 ) ) ;
#15615=EDGE_CURVE ( 'NONE', #101262, #76681, #114177, .T. ) ;
#15616=ORIENTED_EDGE ( 'NONE', *, *, #62860, .F. ) ;
#15617=DIRECTION ( 'NONE',  ( -0.000000000000000000, 1.000000000000000000, -0.000000000000000000 ) ) ;
#15618=DIRECTION ( 'NONE',  ( 0.000000000000000000, -0.000000000000000000, 1.000000000000000000 ) ) ;
#15619=AXIS2_PLACEMENT_3D ( 'NONE', #107721, #88046, #48160 ) ;
#15620=CONICAL_SURFACE ( 'NONE', #72093, 0.1000000000000000472, 0.003490658503988666988 ) ;
#15621=ORIENTED_EDGE ( 'NONE', *, *, #39439, .T. ) ;
#15622=DIRECTION ( 'NONE',  ( 0.000000000000000000, 1.000000000000000000, 0.000000000000000000 ) ) ;
#15623=CARTESIAN_POINT ( 'NONE',  ( 13.14999999999990088, 2.500000000000000000, 1.918653347947321564 ) ) ;
#15624=CARTESIAN_POINT ( 'NONE',  ( 8.749999999999953815, 12.50000000000000000, 6.495190528383297135 ) ) ;
#15626=ORIENTED_EDGE ( 'NONE', *, *, #58628, .T. ) ;
#15627=DIRECTION ( 'NONE',  ( -4.274815082592931898E-19, -0.9999939076577903929, -0.003490651415223739937 ) ) ;
#15628=EDGE_CURVE ( 'NONE', #82756, #72150, #457, .T. ) ;
#15629=VERTEX_POINT ( 'NONE', #113009 ) ;
#15630=CARTESIAN_POINT ( 'NONE',  ( 9.799999999999913669, 2.500000000000000000, -3.983716857408426293 ) ) ;
#15631=DIRECTION ( 'NONE',  ( -0.000000000000000000, 1.000000000000000000, -0.000000000000000000 ) ) ;
#15632=CIRCLE ( 'NONE', #3144, 0.06509327318403741736 ) ;
#15633=EDGE_LOOP ( 'NONE', ( #49898, #64759, #37792, #71767 ) ) ;
#15634=DIRECTION ( 'NONE',  ( -4.274815082592931898E-19, -0.9999939076577903929, -0.003490651415223739937 ) ) ;
#15635=CARTESIAN_POINT ( 'NONE',  ( 6.899999999999928413, 2.500000000000000000, 3.983716857408420964 ) ) ;
#15636=DIRECTION ( 'NONE',  ( -0.000000000000000000, -1.000000000000000000, -0.000000000000000000 ) ) ;
#15637=DIRECTION ( 'NONE',  ( 0.000000000000000000, -0.000000000000000000, 1.000000000000000000 ) ) ;
#15638=DIRECTION ( 'NONE',  ( 0.000000000000000000, 0.000000000000000000, 1.000000000000000000 ) ) ;
#15639=ORIENTED_EDGE ( 'NONE', *, *, #70950, .T. ) ;
#15640=ORIENTED_EDGE ( 'NONE', *, *, #127711, .T. ) ;
#15641=DIRECTION ( 'NONE',  ( 0.000000000000000000, 1.000000000000000000, 0.000000000000000000 ) ) ;
#15642=AXIS2_PLACEMENT_3D ( 'NONE', #87713, #59591, #127649 ) ;
#15643=AXIS2_PLACEMENT_3D ( 'NONE', #40275, #30470, #128683 ) ;
#15644=ADVANCED_FACE ( 'NONE', ( #23326 ), #89130, .T. ) ;
#15646=CARTESIAN_POINT ( 'NONE',  ( -6.650000000000019007, 2.500000000000000000, -5.802370205355749988 ) ) ;
#15647=ORIENTED_EDGE ( 'NONE', *, *, #53263, .T. ) ;
#15648=ORIENTED_EDGE ( 'NONE', *, *, #19886, .T. ) ;
#15649=EDGE_LOOP ( 'NONE', ( #86903, #99261 ) ) ;
#15650=CARTESIAN_POINT ( 'NONE',  ( -3.150000000000030109, 2.500000000000000000, -2.511473670974877948 ) ) ;
#15651=CIRCLE ( 'NONE', #55384, 0.06509327318403745899 ) ;
#15652=CARTESIAN_POINT ( 'NONE',  ( -5.200000000000022382, 12.50000000000000000, 4.741630453620009789 ) ) ;
#15653=CARTESIAN_POINT ( 'NONE',  ( -10.85000000000000142, 2.500000000000000000, -2.265063509461097802 ) ) ;
#15655=DIRECTION ( 'NONE',  ( 0.000000000000000000, 0.000000000000000000, 1.000000000000000000 ) ) ;
#15656=FACE_OUTER_BOUND ( 'NONE', #129183, .T. ) ;
#15657=CARTESIAN_POINT ( 'NONE',  ( 14.99999999999989342, 2.500000000000000000, -0.6928203230275541413 ) ) ;
#15658=DIRECTION ( 'NONE',  ( 0.000000000000000000, 0.000000000000000000, 1.000000000000000000 ) ) ;
#15659=EDGE_CURVE ( 'NONE', #85940, #56105, #84925, .T. ) ;
#15660=DIRECTION ( 'NONE',  ( 0.000000000000000000, -0.9999939076577903929, 0.003490651415223739937 ) ) ;
#15662=AXIS2_PLACEMENT_3D ( 'NONE', #108589, #89598, #81073 ) ;
#15663=AXIS2_PLACEMENT_3D ( 'NONE', #42950, #82859, #73648 ) ;
#15664=DIRECTION ( 'NONE',  ( 0.000000000000000000, 0.000000000000000000, 1.000000000000000000 ) ) ;
#15665=CIRCLE ( 'NONE', #7355, 0.09999999999999982514 ) ;
#15667=ADVANCED_FACE ( 'NONE', ( #4317 ), #76611, .T. ) ;
#15668=EDGE_LOOP ( 'NONE', ( #128274, #81775 ) ) ;
#15669=DIRECTION ( 'NONE',  ( 0.000000000000000000, 1.000000000000000000, 0.000000000000000000 ) ) ;
#15670=DIRECTION ( 'NONE',  ( -0.000000000000000000, 1.000000000000000000, -0.000000000000000000 ) ) ;
#15671=CARTESIAN_POINT ( 'NONE',  ( 12.69999999999990337, 2.500000000000000000, -4.676537180435978769 ) ) ;
#15672=CIRCLE ( 'NONE', #74187, 0.1000000000000002554 ) ;
#15673=CARTESIAN_POINT ( 'NONE',  ( -3.750000000000025757, 2.500000000000000000, -2.857883832488653741 ) ) ;
#15674=AXIS2_PLACEMENT_3D ( 'NONE', #102101, #82473, #22905 ) ;
#15675=CIRCLE ( 'NONE', #9445, 0.1000000000000002554 ) ;
#15676=DIRECTION ( 'NONE',  ( -0.000000000000000000, 1.000000000000000000, -0.000000000000000000 ) ) ;
#15677=LINE ( 'NONE', #117097, #124357 ) ;
#15678=DIRECTION ( 'NONE',  ( 0.000000000000000000, 0.000000000000000000, 1.000000000000000000 ) ) ;
#15679=EDGE_LOOP ( 'NONE', ( #16231, #12473, #72538, #26577 ) ) ;
#15680=DIRECTION ( 'NONE',  ( 0.000000000000000000, 1.000000000000000000, 0.000000000000000000 ) ) ;
#15681=AXIS2_PLACEMENT_3D ( 'NONE', #114401, #24098, #103949 ) ;
#15682=FACE_OUTER_BOUND ( 'NONE', #69945, .T. ) ;
#15683=CONICAL_SURFACE ( 'NONE', #97267, 0.09999999999999999167, 0.003490658503988666988 ) ;
#15684=ORIENTED_EDGE ( 'NONE', *, *, #82068, .T. ) ;
#15685=VECTOR ( 'NONE', #111584, 1000.000000000000000 ) ;
#15686=EDGE_LOOP ( 'NONE', ( #90829, #39291, #43700, #65240 ) ) ;
#15687=ADVANCED_FACE ( 'NONE', ( #124114 ), #105859, .T. ) ;
#15688=EDGE_LOOP ( 'NONE', ( #55524, #35214, #24544, #51695 ) ) ;
#15689=VECTOR ( 'NONE', #95081, 1000.000000000000000 ) ;
#15690=ORIENTED_EDGE ( 'NONE', *, *, #23388, .F. ) ;
#15691=DIRECTION ( 'NONE',  ( 0.000000000000000000, 0.000000000000000000, 1.000000000000000000 ) ) ;
#15692=CARTESIAN_POINT ( 'NONE',  ( -9.350000000000008527, 2.500000000000000000, -6.048780366869521252 ) ) ;
#15693=ADVANCED_FACE ( 'NONE', ( #83566 ), #39078, .T. ) ;
#15694=CARTESIAN_POINT ( 'NONE',  ( -10.20000000000000284, 2.500000000000000000, 4.083716857408421497 ) ) ;
#15695=CARTESIAN_POINT ( 'NONE',  ( -9.999999999999971578, 2.500000000000000000, -4.330127018922197202 ) ) ;
#15696=DIRECTION ( 'NONE',  ( -0.000000000000000000, -1.000000000000000000, -0.000000000000000000 ) ) ;
#15697=VERTEX_POINT ( 'NONE', #64549 ) ;
#15698=CARTESIAN_POINT ( 'NONE',  ( -14.14999999999998792, 2.500000000000000000, -1.372243186433547812 ) ) ;
#15700=EDGE_CURVE ( 'NONE', #90750, #72456, #44926, .T. ) ;
#15701=EDGE_CURVE ( 'NONE', #26026, #108711, #104473, .T. ) ;
#15702=DIRECTION ( 'NONE',  ( -4.274815082592931898E-19, -0.9999939076577903929, -0.003490651415223739937 ) ) ;
#15703=EDGE_CURVE ( 'NONE', #74853, #52514, #82920, .T. ) ;
#15704=AXIS2_PLACEMENT_3D ( 'NONE', #102253, #43340, #64245 ) ;
#15706=ORIENTED_EDGE ( 'NONE', *, *, #39245, .F. ) ;
#15707=VERTEX_POINT ( 'NONE', #55385 ) ;
#15708=ADVANCED_FACE ( 'NONE', ( #95309 ), #12850, .T. ) ;
#15709=ORIENTED_EDGE ( 'NONE', *, *, #26631, .T. ) ;
#15710=LINE ( 'NONE', #106043, #105216 ) ;
#15711=EDGE_CURVE ( 'NONE', #56932, #106131, #47369, .T. ) ;
#15712=AXIS2_PLACEMENT_3D ( 'NONE', #24977, #16413, #33526 ) ;
#15713=EDGE_CURVE ( 'NONE', #56340, #19273, #110066, .T. ) ;
#15714=AXIS2_PLACEMENT_3D ( 'NONE', #8221, #19996, #128004 ) ;
#15715=FACE_OUTER_BOUND ( 'NONE', #36806, .T. ) ;
#15716=DIRECTION ( 'NONE',  ( 0.000000000000000000, 1.000000000000000000, 0.000000000000000000 ) ) ;
#15717=CONICAL_SURFACE ( 'NONE', #97305, 0.09999999999999982514, 0.003490658503988666988 ) ;
#15718=EDGE_CURVE ( 'NONE', #128284, #57396, #93376, .T. ) ;
#15720=EDGE_LOOP ( 'NONE', ( #42680, #116032, #58088, #74123 ) ) ;
#15721=DIRECTION ( 'NONE',  ( 0.000000000000000000, 0.000000000000000000, 1.000000000000000000 ) ) ;
#15722=FACE_OUTER_BOUND ( 'NONE', #1280, .T. ) ;
#15723=DIRECTION ( 'NONE',  ( 0.000000000000000000, 1.000000000000000000, 0.000000000000000000 ) ) ;
#15724=DIRECTION ( 'NONE',  ( 0.000000000000000000, 1.000000000000000000, 0.000000000000000000 ) ) ;
#15725=DIRECTION ( 'NONE',  ( 0.000000000000000000, 0.000000000000000000, 1.000000000000000000 ) ) ;
#15726=ADVANCED_FACE ( 'NONE', ( #5614 ), #33185, .T. ) ;
#15727=AXIS2_PLACEMENT_3D ( 'NONE', #91734, #2050, #52445 ) ;
#15728=EDGE_LOOP ( 'NONE', ( #126427, #27391, #49551, #43110 ) ) ;
#15729=CARTESIAN_POINT ( 'NONE',  ( -2.950000000000029932, 12.50000000000000000, 2.165063509461097713 ) ) ;
#15730=CIRCLE ( 'NONE', #36691, 0.06509327318403745899 ) ;
#15732=ORIENTED_EDGE ( 'NONE', *, *, #50306, .T. ) ;
#15733=EDGE_LOOP ( 'NONE', ( #89097, #97240, #94497, #29643 ) ) ;
#15734=CARTESIAN_POINT ( 'NONE',  ( -5.400000000000019895, 12.50000000000000000, -0.6928203230275541413 ) ) ;
#15735=FACE_BOUND ( 'NONE', #15188, .T. ) ;
#15736=DIRECTION ( 'NONE',  ( -0.000000000000000000, -1.000000000000000000, -0.000000000000000000 ) ) ;
#15737=DIRECTION ( 'NONE',  ( 0.000000000000000000, 0.000000000000000000, -1.000000000000000000 ) ) ;
#15738=CARTESIAN_POINT ( 'NONE',  ( -9.550000000000007816, 2.500000000000000000, -6.495190528383297135 ) ) ;
#15739=CIRCLE ( 'NONE', #109757, 0.1000000000000000472 ) ;
#15740=VECTOR ( 'NONE', #44791, 1000.000000000000000 ) ;
#15741=ORIENTED_EDGE ( 'NONE', *, *, #102292, .T. ) ;
#15742=CARTESIAN_POINT ( 'NONE',  ( 6.849999999999929479, 2.500000000000000000, -2.511473670974877948 ) ) ;
#15743=DIRECTION ( 'NONE',  ( 0.000000000000000000, 1.000000000000000000, 0.000000000000000000 ) ) ;
#15744=DIRECTION ( 'NONE',  ( 0.000000000000000000, 1.000000000000000000, 0.000000000000000000 ) ) ;
#15745=FACE_OUTER_BOUND ( 'NONE', #23040, .T. ) ;
#15746=ORIENTED_EDGE ( 'NONE', *, *, #74394, .F. ) ;
#15747=CARTESIAN_POINT ( 'NONE',  ( 11.44999999999990514, 2.500000000000000000, -6.248780366869526759 ) ) ;
#15748=FACE_OUTER_BOUND ( 'NONE', #35338, .T. ) ;
#15750=ORIENTED_EDGE ( 'NONE', *, *, #74186, .T. ) ;
#15751=CARTESIAN_POINT ( 'NONE',  ( 6.649999999999927525, 12.50000000000000000, 2.165063509461097713 ) ) ;
#15752=CIRCLE ( 'NONE', #88938, 0.09999999999999982514 ) ;
#15753=ORIENTED_EDGE ( 'NONE', *, *, #100391, .F. ) ;
#15754=FACE_BOUND ( 'NONE', #90528, .T. ) ;
#15755=CARTESIAN_POINT ( 'NONE',  ( -8.300000000000011369, 2.500000000000000000, -4.330127018922201643 ) ) ;
#15756=EDGE_CURVE ( 'NONE', #82926, #120749, #103842, .T. ) ;
#15757=CIRCLE ( 'NONE', #3173, 0.06509327318403743123 ) ;
#15758=ORIENTED_EDGE ( 'NONE', *, *, #2345, .F. ) ;
#15759=FACE_OUTER_BOUND ( 'NONE', #76218, .T. ) ;
#15760=DIRECTION ( 'NONE',  ( 0.000000000000000000, 1.000000000000000000, 0.000000000000000000 ) ) ;
#15761=AXIS2_PLACEMENT_3D ( 'NONE', #46621, #15865, #86546 ) ;
#15762=EDGE_CURVE ( 'NONE', #79929, #24152, #18111, .T. ) ;
#15763=EDGE_LOOP ( 'NONE', ( #23908, #80187, #59821, #56332 ) ) ;
#15765=ORIENTED_EDGE ( 'NONE', *, *, #76416, .T. ) ;
#15767=ORIENTED_EDGE ( 'NONE', *, *, #105524, .T. ) ;
#15769=CARTESIAN_POINT ( 'NONE',  ( -11.64999999999999858, 2.500000000000000000, -1.372243186433546036 ) ) ;
#15770=AXIS2_PLACEMENT_3D ( 'NONE', #82681, #94400, #55774 ) ;
#15771=ADVANCED_FACE ( 'NONE', ( #116222 ), #128957, .T. ) ;
#15772=CIRCLE ( 'NONE', #76340, 0.1000000000000000472 ) ;
#15773=CARTESIAN_POINT ( 'NONE',  ( 0.4499999999999569344, 2.500000000000000000, -2.165063509461101710 ) ) ;
#15774=CARTESIAN_POINT ( 'NONE',  ( 5.849999999999935696, 2.500000000000000000, -7.288010851410854585 ) ) ;
#15775=AXIS2_PLACEMENT_3D ( 'NONE', #82876, #3018, #42972 ) ;
#15776=DIRECTION ( 'NONE',  ( 0.000000000000000000, 0.000000000000000000, 1.000000000000000000 ) ) ;
#15777=VECTOR ( 'NONE', #20063, 1000.000000000000000 ) ;
#15778=AXIS2_PLACEMENT_3D ( 'NONE', #19157, #69563, #68270 ) ;
#15779=ORIENTED_EDGE ( 'NONE', *, *, #106575, .F. ) ;
#15780=ORIENTED_EDGE ( 'NONE', *, *, #95880, .T. ) ;
#15781=CARTESIAN_POINT ( 'NONE',  ( -9.400000000000009237, 2.500000000000000000, -3.983716857408421852 ) ) ;
#15782=CARTESIAN_POINT ( 'NONE',  ( -11.44999999999999751, 2.500000000000000000, 2.511473670974873507 ) ) ;
#15783=DIRECTION ( 'NONE',  ( 0.000000000000000000, 1.000000000000000000, 0.000000000000000000 ) ) ;
#15784=AXIS2_PLACEMENT_3D ( 'NONE', #72708, #121159, #52415 ) ;
#15785=LINE ( 'NONE', #55717, #78293 ) ;
#15786=ORIENTED_EDGE ( 'NONE', *, *, #48643, .T. ) ;
#15787=EDGE_LOOP ( 'NONE', ( #122378, #15044, #12079, #28384 ) ) ;
#15788=PLANE ( 'NONE',  #95543 ) ;
#15789=ORIENTED_EDGE ( 'NONE', *, *, #1251, .F. ) ;
#15790=CARTESIAN_POINT ( 'NONE',  ( -14.14999999999998614, 2.500000000000000000, 2.165063509461101265 ) ) ;
#15791=DIRECTION ( 'NONE',  ( 0.000000000000000000, 1.000000000000000000, 0.000000000000000000 ) ) ;
#15792=VERTEX_POINT ( 'NONE', #6255 ) ;
#15793=CARTESIAN_POINT ( 'NONE',  ( -14.59999999999998366, 12.50000000000000000, -0.6277270498435145729 ) ) ;
#15794=CARTESIAN_POINT ( 'NONE',  ( 14.59999999999989484, 12.50000000000000000, -0.6928203230275541413 ) ) ;
#15795=CARTESIAN_POINT ( 'NONE',  ( -1.050000000000037348, 2.500000000000000000, -2.411473670974877859 ) ) ;
#15796=LINE ( 'NONE', #97586, #52847 ) ;
#15798=FACE_OUTER_BOUND ( 'NONE', #58359, .T. ) ;
#15799=DIRECTION ( 'NONE',  ( 0.000000000000000000, 0.000000000000000000, 1.000000000000000000 ) ) ;
#15800=DIRECTION ( 'NONE',  ( 0.000000000000000000, 0.000000000000000000, -1.000000000000000000 ) ) ;
#15801=DIRECTION ( 'NONE',  ( 0.000000000000000000, 0.000000000000000000, -1.000000000000000000 ) ) ;
#15802=ADVANCED_FACE ( 'NONE', ( #48627 ), #30295, .T. ) ;
#15803=ORIENTED_EDGE ( 'NONE', *, *, #124543, .T. ) ;
#15806=ORIENTED_EDGE ( 'NONE', *, *, #73936, .T. ) ;
#15807=LINE ( 'NONE', #7923, #89581 ) ;
#15808=EDGE_LOOP ( 'NONE', ( #27171, #52875 ) ) ;
#15809=ORIENTED_EDGE ( 'NONE', *, *, #75036, .T. ) ;
#15811=ORIENTED_EDGE ( 'NONE', *, *, #128860, .T. ) ;
#15812=EDGE_CURVE ( 'NONE', #74379, #89315, #120529, .T. ) ;
#15813=FACE_OUTER_BOUND ( 'NONE', #4161, .T. ) ;
#15814=AXIS2_PLACEMENT_3D ( 'NONE', #72929, #42859, #112215 ) ;
#15815=CONICAL_SURFACE ( 'NONE', #74413, 0.1000000000000000472, 0.003490658503988666988 ) ;
#15816=FACE_OUTER_BOUND ( 'NONE', #77293, .T. ) ;
#15817=CONICAL_SURFACE ( 'NONE', #122451, 0.1000000000000002554, 0.003490658503988666988 ) ;
#15818=CARTESIAN_POINT ( 'NONE',  ( 8.099999999999921485, 2.500000000000000000, 0.4464101615137735513 ) ) ;
#15819=CARTESIAN_POINT ( 'NONE',  ( 0.6499999999999566125, 12.50000000000000000, -6.906693963081115051 ) ) ;
#15820=EDGE_CURVE ( 'NONE', #86126, #27663, #112211, .T. ) ;
#15821=DIRECTION ( 'NONE',  ( -0.000000000000000000, -1.000000000000000000, -0.000000000000000000 ) ) ;
#15822=VERTEX_POINT ( 'NONE', #9342 ) ;
#15823=ADVANCED_FACE ( 'NONE', ( #128499 ), #101746, .T. ) ;
#15824=CARTESIAN_POINT ( 'NONE',  ( 8.749999999999921840, 12.50000000000000000, 2.922977105672686982 ) ) ;
#15825=ORIENTED_EDGE ( 'NONE', *, *, #129082, .T. ) ;
#15826=CIRCLE ( 'NONE', #43058, 0.06509327318403745899 ) ;
#15827=EDGE_LOOP ( 'NONE', ( #36784, #25222, #64296, #33244 ) ) ;
#15828=ORIENTED_EDGE ( 'NONE', *, *, #83091, .F. ) ;
#15829=EDGE_LOOP ( 'NONE', ( #849, #79661 ) ) ;
#15830=AXIS2_PLACEMENT_3D ( 'NONE', #121743, #104049, #13716 ) ;
#15831=AXIS2_PLACEMENT_3D ( 'NONE', #22742, #22097, #11607 ) ;
#15833=ORIENTED_EDGE ( 'NONE', *, *, #52360, .F. ) ;
#15834=EDGE_CURVE ( 'NONE', #107252, #87657, #97527, .T. ) ;
#15835=ORIENTED_EDGE ( 'NONE', *, *, #36588, .T. ) ;
#15836=DIRECTION ( 'NONE',  ( -4.274815082592931898E-19, -0.9999939076577903929, -0.003490651415223739937 ) ) ;
#15837=FACE_OUTER_BOUND ( 'NONE', #79505, .T. ) ;
#15838=AXIS2_PLACEMENT_3D ( 'NONE', #42183, #52634, #2904 ) ;
#15839=CARTESIAN_POINT ( 'NONE',  ( -5.800000000000018474, 2.500000000000000000, -2.276824562219559311E-15 ) ) ;
#15840=CIRCLE ( 'NONE', #89016, 0.09999999999999982514 ) ;
#15841=DIRECTION ( 'NONE',  ( 0.000000000000000000, 1.000000000000000000, 0.000000000000000000 ) ) ;
#15842=CARTESIAN_POINT ( 'NONE',  ( 1.049999999999953637, 2.500000000000000000, 2.411473670974873862 ) ) ;
#15843=DIRECTION ( 'NONE',  ( -0.000000000000000000, -1.000000000000000000, -0.000000000000000000 ) ) ;
#15844=EDGE_LOOP ( 'NONE', ( #52282, #62267 ) ) ;
#15845=CARTESIAN_POINT ( 'NONE',  ( -4.150000000000027889, 2.500000000000000000, -7.288010851410854585 ) ) ;
#15846=VERTEX_POINT ( 'NONE', #49936 ) ;
#15847=CARTESIAN_POINT ( 'NONE',  ( -12.89999999999999147, 2.500000000000000000, -0.5928203230275499447 ) ) ;
#15848=ORIENTED_EDGE ( 'NONE', *, *, #106173, .T. ) ;
#15849=DIRECTION ( 'NONE',  ( -0.000000000000000000, 1.000000000000000000, -0.000000000000000000 ) ) ;
#15850=ORIENTED_EDGE ( 'NONE', *, *, #114069, .F. ) ;
#15851=ORIENTED_EDGE ( 'NONE', *, *, #46651, .F. ) ;
#15852=DIRECTION ( 'NONE',  ( 0.000000000000000000, -0.9999939076577903929, 0.003490651415223739937 ) ) ;
#15853=FACE_OUTER_BOUND ( 'NONE', #34533, .T. ) ;
#15854=ADVANCED_FACE ( 'NONE', ( #60400 ), #28593, .T. ) ;
#15855=CIRCLE ( 'NONE', #1199, 0.06509327318403745899 ) ;
#15857=AXIS2_PLACEMENT_3D ( 'NONE', #108755, #97656, #127137 ) ;
#15858=DIRECTION ( 'NONE',  ( -0.000000000000000000, -1.000000000000000000, -0.000000000000000000 ) ) ;
#15859=CARTESIAN_POINT ( 'NONE',  ( 9.349999999999919709, 2.500000000000000000, 1.818653347947321475 ) ) ;
#15860=ORIENTED_EDGE ( 'NONE', *, *, #78097, .F. ) ;
#15861=DIRECTION ( 'NONE',  ( 0.000000000000000000, 0.000000000000000000, 1.000000000000000000 ) ) ;
#15862=DIRECTION ( 'NONE',  ( 0.000000000000000000, 0.000000000000000000, 1.000000000000000000 ) ) ;
#15863=EDGE_CURVE ( 'NONE', #98343, #35123, #89829, .T. ) ;
#15865=DIRECTION ( 'NONE',  ( 0.000000000000000000, 1.000000000000000000, 0.000000000000000000 ) ) ;
#15866=ADVANCED_FACE ( 'NONE', ( #115568 ), #45324, .T. ) ;
#15867=CARTESIAN_POINT ( 'NONE',  ( -3.350000000000028955, 2.500000000000000000, -2.165063509461101710 ) ) ;
#15868=ORIENTED_EDGE ( 'NONE', *, *, #50464, .F. ) ;
#15869=VERTEX_POINT ( 'NONE', #25930 ) ;
#15870=ADVANCED_FACE ( 'NONE', ( #110121 ), #1384, .T. ) ;
#15871=CIRCLE ( 'NONE', #7460, 0.06509327318403745899 ) ;
#15872=EDGE_CURVE ( 'NONE', #111323, #4351, #62046, .T. ) ;
#15873=ADVANCED_FACE ( 'NONE', ( #40096 ), #87061, .T. ) ;
#15874=ORIENTED_EDGE ( 'NONE', *, *, #129252, .T. ) ;
#15875=VECTOR ( 'NONE', #111491, 1000.000000000000000 ) ;
#15876=LINE ( 'NONE', #56444, #125990 ) ;
#15877=DIRECTION ( 'NONE',  ( 0.000000000000000000, 0.000000000000000000, -1.000000000000000000 ) ) ;
#15878=AXIS2_PLACEMENT_3D ( 'NONE', #112727, #2758, #82629 ) ;
#15879=AXIS2_PLACEMENT_3D ( 'NONE', #6615, #36779, #20347 ) ;
#15880=ADVANCED_FACE ( 'NONE', ( #95948 ), #114255, .T. ) ;
#15881=CONICAL_SURFACE ( 'NONE', #91107, 0.1000000000000002554, 0.003490658503988666988 ) ;
#15883=DIRECTION ( 'NONE',  ( 0.000000000000000000, 0.000000000000000000, 1.000000000000000000 ) ) ;
#15884=CARTESIAN_POINT ( 'NONE',  ( 2.699999999999945555, 12.50000000000000000, 3.983716857408420076 ) ) ;
#15885=CARTESIAN_POINT ( 'NONE',  ( -1.250000000000036193, 2.500000000000000000, 5.802370205355744659 ) ) ;
#15886=DIRECTION ( 'NONE',  ( -4.274815082592931898E-19, -0.9999939076577903929, -0.003490651415223739937 ) ) ;
#15887=VERTEX_POINT ( 'NONE', #28995 ) ;
#15888=ADVANCED_FACE ( 'NONE', ( #99666 ), #34870, .T. ) ;
#15889=DIRECTION ( 'NONE',  ( 0.000000000000000000, 0.000000000000000000, 1.000000000000000000 ) ) ;
#15890=CARTESIAN_POINT ( 'NONE',  ( 3.149999999999942624, 12.50000000000000000, 6.906693963081109722 ) ) ;
#15891=ORIENTED_EDGE ( 'NONE', *, *, #43119, .T. ) ;
#15892=FACE_OUTER_BOUND ( 'NONE', #100368, .T. ) ;
#15893=CARTESIAN_POINT ( 'NONE',  ( 2.499999999999948930, 2.500000000000000000, -4.922947341949753586 ) ) ;
#15894=DIRECTION ( 'NONE',  ( 0.000000000000000000, 1.000000000000000000, 0.000000000000000000 ) ) ;
#15895=ORIENTED_EDGE ( 'NONE', *, *, #86961, .T. ) ;
#15896=CARTESIAN_POINT ( 'NONE',  ( 5.399999999999936406, 2.500000000000000000, -5.022947341949754119 ) ) ;
#15897=CONICAL_SURFACE ( 'NONE', #84954, 0.09999999999999982514, 0.003490658503988666988 ) ;
#15898=ORIENTED_EDGE ( 'NONE', *, *, #88906, .F. ) ;
#15899=DIRECTION ( 'NONE',  ( -0.000000000000000000, -1.000000000000000000, -0.000000000000000000 ) ) ;
#15900=CARTESIAN_POINT ( 'NONE',  ( -6.450000000000017941, 12.50000000000000000, -2.511473670974877948 ) ) ;
#15901=AXIS2_PLACEMENT_3D ( 'NONE', #43329, #13187, #123168 ) ;
#15902=AXIS2_PLACEMENT_3D ( 'NONE', #41403, #81314, #23674 ) ;
#15903=VERTEX_POINT ( 'NONE', #125410 ) ;
#15904=CARTESIAN_POINT ( 'NONE',  ( -5.650000000000019895, 12.50000000000000000, 1.818653347947321475 ) ) ;
#15905=AXIS2_PLACEMENT_3D ( 'NONE', #120424, #31409, #30774 ) ;
#15906=DIRECTION ( 'NONE',  ( 0.000000000000000000, 1.000000000000000000, 0.000000000000000000 ) ) ;
#15907=VERTEX_POINT ( 'NONE', #58458 ) ;
#15908=FACE_OUTER_BOUND ( 'NONE', #41058, .T. ) ;
#15909=VECTOR ( 'NONE', #67237, 1000.000000000000000 ) ;
#15910=ADVANCED_FACE ( 'NONE', ( #68899 ), #60007, .T. ) ;
#15911=ORIENTED_EDGE ( 'NONE', *, *, #110716, .T. ) ;
#15912=ORIENTED_EDGE ( 'NONE', *, *, #5363, .F. ) ;
#15913=CARTESIAN_POINT ( 'NONE',  ( 3.099999999999945022, 12.50000000000000000, -4.676537180435978769 ) ) ;
#15914=LINE ( 'NONE', #23163, #62593 ) ;
#15915=VERTEX_POINT ( 'NONE', #21088 ) ;
#15916=DIRECTION ( 'NONE',  ( 0.000000000000000000, 1.000000000000000000, 0.000000000000000000 ) ) ;
#15917=DIRECTION ( 'NONE',  ( 0.000000000000000000, 0.000000000000000000, -1.000000000000000000 ) ) ;
#15918=ORIENTED_EDGE ( 'NONE', *, *, #125521, .F. ) ;
#15919=EDGE_CURVE ( 'NONE', #123777, #115296, #105945, .T. ) ;
#15920=CARTESIAN_POINT ( 'NONE',  ( 10.44999999999991402, 12.50000000000000000, 6.495190528383297135 ) ) ;
#15921=DIRECTION ( 'NONE',  ( -0.000000000000000000, 1.000000000000000000, -0.000000000000000000 ) ) ;
#15922=CARTESIAN_POINT ( 'NONE',  ( -3.350000000000028511, 12.50000000000000000, 2.857883832488649301 ) ) ;
#15923=FACE_OUTER_BOUND ( 'NONE', #89774, .T. ) ;
#15924=CARTESIAN_POINT ( 'NONE',  ( -6.505213034913026604E-15, 12.50000000000000000, 4.330127018922196314 ) ) ;
#15925=DIRECTION ( 'NONE',  ( 0.000000000000000000, 0.000000000000000000, 1.000000000000000000 ) ) ;
#15926=VERTEX_POINT ( 'NONE', #10604 ) ;
#15927=ORIENTED_EDGE ( 'NONE', *, *, #73766, .F. ) ;
#15928=EDGE_LOOP ( 'NONE', ( #19221, #52078 ) ) ;
#15929=ORIENTED_EDGE ( 'NONE', *, *, #94768, .T. ) ;
#15930=CARTESIAN_POINT ( 'NONE',  ( 76.44220535185989718, 3.905138931494375854, 5.869652189505977447 ) ) ;
#15931=DIRECTION ( 'NONE',  ( 0.000000000000000000, 1.000000000000000000, 0.000000000000000000 ) ) ;
#15932=DIRECTION ( 'NONE',  ( -0.000000000000000000, 1.000000000000000000, -0.000000000000000000 ) ) ;
#15933=VERTEX_POINT ( 'NONE', #21747 ) ;
#15934=FACE_BOUND ( 'NONE', #23210, .T. ) ;
#15935=FACE_OUTER_BOUND ( 'NONE', #71650, .T. ) ;
#15936=DIRECTION ( 'NONE',  ( 0.000000000000000000, -0.000000000000000000, 1.000000000000000000 ) ) ;
#15937=LINE ( 'NONE', #5476, #32465 ) ;
#15938=VECTOR ( 'NONE', #21117, 1000.000000000000000 ) ;
#15939=DIRECTION ( 'NONE',  ( 0.000000000000000000, 1.000000000000000000, 0.000000000000000000 ) ) ;
#15940=CONICAL_SURFACE ( 'NONE', #91266, 0.09999999999999982514, 0.003490658503988666988 ) ;
#15941=CARTESIAN_POINT ( 'NONE',  ( 1.449999999999951328, 2.500000000000000000, 2.611473670974873151 ) ) ;
#15942=LINE ( 'NONE', #108202, #108222 ) ;
#15943=CARTESIAN_POINT ( 'NONE',  ( 5.199999999999933564, 2.500000000000000000, 0.2464101615137735679 ) ) ;
#15944=FACE_OUTER_BOUND ( 'NONE', #58506, .T. ) ;
#15945=DIRECTION ( 'NONE',  ( 0.000000000000000000, 1.000000000000000000, 0.000000000000000000 ) ) ;
#15946=CARTESIAN_POINT ( 'NONE',  ( -1.250000000000001554, 2.500000000000000000, 2.165063509461097713 ) ) ;
#15947=AXIS2_PLACEMENT_3D ( 'NONE', #19924, #22514, #41513 ) ;
#15948=AXIS2_PLACEMENT_3D ( 'NONE', #99981, #49603, #59431 ) ;
#15949=EDGE_CURVE ( 'NONE', #70884, #78664, #12548, .T. ) ;
#15950=VERTEX_POINT ( 'NONE', #40763 ) ;
#15951=ORIENTED_EDGE ( 'NONE', *, *, #6828, .F. ) ;
#15952=EDGE_LOOP ( 'NONE', ( #40600, #55313 ) ) ;
#15953=ORIENTED_EDGE ( 'NONE', *, *, #106364, .T. ) ;
#15954=CARTESIAN_POINT ( 'NONE',  ( 11.24999999999990585, 2.500000000000000000, 2.757883832488649656 ) ) ;
#15955=VERTEX_POINT ( 'NONE', #1446 ) ;
#15956=DIRECTION ( 'NONE',  ( 0.000000000000000000, -0.000000000000000000, 1.000000000000000000 ) ) ;
#15957=ORIENTED_EDGE ( 'NONE', *, *, #81790, .T. ) ;
#15958=VERTEX_POINT ( 'NONE', #32228 ) ;
#15959=CARTESIAN_POINT ( 'NONE',  ( 5.649999999999934630, 2.500000000000000000, -2.511473670974877948 ) ) ;
#15960=CONICAL_SURFACE ( 'NONE', #9622, 0.1000000000000002554, 0.003490658503988666988 ) ;
#15961=AXIS2_PLACEMENT_3D ( 'NONE', #85782, #73387, #55046 ) ;
#15962=EDGE_CURVE ( 'NONE', #109761, #55194, #90461, .T. ) ;
#15963=AXIS2_PLACEMENT_3D ( 'NONE', #54950, #111958, #83771 ) ;
#15964=DIRECTION ( 'NONE',  ( -0.000000000000000000, -1.000000000000000000, -0.000000000000000000 ) ) ;
#15965=DIRECTION ( 'NONE',  ( 0.000000000000000000, -0.9999939076577903929, 0.003490651415223739937 ) ) ;
#15966=CARTESIAN_POINT ( 'NONE',  ( 1.899999999999951283, 12.50000000000000000, 0.3464101615137736845 ) ) ;
#15967=DIRECTION ( 'NONE',  ( 0.000000000000000000, 1.000000000000000000, 0.000000000000000000 ) ) ;
#15968=EDGE_CURVE ( 'NONE', #95053, #41415, #122667, .T. ) ;
#15969=EDGE_CURVE ( 'NONE', #4541, #94964, #99699, .T. ) ;
#15970=ORIENTED_EDGE ( 'NONE', *, *, #98280, .T. ) ;
#15971=ORIENTED_EDGE ( 'NONE', *, *, #122295, .T. ) ;
#15972=ORIENTED_EDGE ( 'NONE', *, *, #114552, .T. ) ;
#15973=ORIENTED_EDGE ( 'NONE', *, *, #70124, .T. ) ;
#15974=EDGE_CURVE ( 'NONE', #129526, #40642, #76702, .T. ) ;
#15975=CARTESIAN_POINT ( 'NONE',  ( -0.8500000000000382805, 12.50000000000000000, -1.472243186433550122 ) ) ;
#15976=ORIENTED_EDGE ( 'NONE', *, *, #27397, .T. ) ;
#15977=EDGE_CURVE ( 'NONE', #51555, #104463, #52478, .T. ) ;
#15978=CIRCLE ( 'NONE', #91220, 0.06509327318403745899 ) ;
#15979=EDGE_LOOP ( 'NONE', ( #22232, #83040, #67763, #21075 ) ) ;
#15980=DIRECTION ( 'NONE',  ( -4.274815082592931898E-19, -0.9999939076577903929, -0.003490651415223739937 ) ) ;
#15981=FACE_OUTER_BOUND ( 'NONE', #127035, .T. ) ;
#15982=PLANE ( 'NONE',  #106346 ) ;
#15983=AXIS2_PLACEMENT_3D ( 'NONE', #59892, #107680, #58589 ) ;
#15984=LINE ( 'NONE', #14049, #106799 ) ;
#15985=CARTESIAN_POINT ( 'NONE',  ( 1.249999999999953815, 2.500000000000000000, 1.572243186433545548 ) ) ;
#15986=CIRCLE ( 'NONE', #32758, 0.06509327318403745899 ) ;
#15987=DIRECTION ( 'NONE',  ( 0.000000000000000000, 0.000000000000000000, 1.000000000000000000 ) ) ;
#15988=VECTOR ( 'NONE', #4643, 1000.000000000000000 ) ;
#15989=ORIENTED_EDGE ( 'NONE', *, *, #37928, .F. ) ;
#15990=DIRECTION ( 'NONE',  ( -0.000000000000000000, -1.000000000000000000, -0.000000000000000000 ) ) ;
#15991=CONICAL_SURFACE ( 'NONE', #76560, 0.1000000000000002554, 0.003490658503988666988 ) ;
#15992=VERTEX_POINT ( 'NONE', #100929 ) ;
#15993=AXIS2_PLACEMENT_3D ( 'NONE', #92236, #23499, #3232 ) ;
#15995=ORIENTED_EDGE ( 'NONE', *, *, #45900, .F. ) ;
#15997=ADVANCED_FACE ( 'NONE', ( #81311 ), #62143, .T. ) ;
#15998=CARTESIAN_POINT ( 'NONE',  ( 4.549999999999939426, 12.50000000000000000, -2.099970236277064473 ) ) ;
#15999=ORIENTED_EDGE ( 'NONE', *, *, #71459, .T. ) ;
#16000=DIRECTION ( 'NONE',  ( -4.274815082592931898E-19, -0.9999939076577903929, -0.003490651415223739937 ) ) ;
#16001=DIRECTION ( 'NONE',  ( 0.000000000000000000, 0.000000000000000000, 1.000000000000000000 ) ) ;
#16002=ORIENTED_EDGE ( 'NONE', *, *, #63499, .T. ) ;
#16003=CIRCLE ( 'NONE', #124694, 0.09999999999999982514 ) ;
#16004=( LENGTH_UNIT ( ) NAMED_UNIT ( * ) SI_UNIT ( .MILLI., .METRE. ) );
#16005=EDGE_CURVE ( 'NONE', #42689, #83000, #97629, .T. ) ;
#16007=AXIS2_PLACEMENT_3D ( 'NONE', #53793, #62344, #12571 ) ;
#16008=CARTESIAN_POINT ( 'NONE',  ( 9.549999999999918998, 2.500000000000000000, 2.265063509461097357 ) ) ;
#16009=ORIENTED_EDGE ( 'NONE', *, *, #69957, .T. ) ;
#16010=ORIENTED_EDGE ( 'NONE', *, *, #84897, .T. ) ;
#16012=CARTESIAN_POINT ( 'NONE',  ( -13.94999999999998685, 12.50000000000000000, 1.818653347947325472 ) ) ;
#16014=CARTESIAN_POINT ( 'NONE',  ( 2.949999999999945111, 2.500000000000000000, 2.165063509461097713 ) ) ;
#16015=EDGE_CURVE ( 'NONE', #76654, #71376, #41222, .T. ) ;
#16017=CARTESIAN_POINT ( 'NONE',  ( -3.350000000000028955, 2.500000000000000000, 2.165063509461097713 ) ) ;
#16018=ADVANCED_FACE ( 'NONE', ( #50540 ), #51855, .T. ) ;
#16020=ADVANCED_FACE ( 'NONE', ( #53139 ), #18198, .T. ) ;
#16021=ORIENTED_EDGE ( 'NONE', *, *, #82925, .T. ) ;
#16022=DIRECTION ( 'NONE',  ( 0.000000000000000000, 1.000000000000000000, 0.000000000000000000 ) ) ;
#16023=ORIENTED_EDGE ( 'NONE', *, *, #87266, .F. ) ;
#16024=EDGE_CURVE ( 'NONE', #107957, #108388, #37093, .T. ) ;
#16025=CARTESIAN_POINT ( 'NONE',  ( 0.6499999999999566125, 2.500000000000000000, -6.148780366869526226 ) ) ;
#16026=DIRECTION ( 'NONE',  ( 0.000000000000000000, 0.000000000000000000, 1.000000000000000000 ) ) ;
#16027=CARTESIAN_POINT ( 'NONE',  ( -9.150000000000005684, 2.500000000000000000, 6.395190528383296602 ) ) ;
#16028=ORIENTED_EDGE ( 'NONE', *, *, #73669, .F. ) ;
#16029=EDGE_CURVE ( 'NONE', #117308, #7829, #91371, .T. ) ;
#16031=AXIS2_PLACEMENT_3D ( 'NONE', #60279, #111254, #10492 ) ;
#16032=CIRCLE ( 'NONE', #3442, 0.06509327318403745899 ) ;
#16033=LINE ( 'NONE', #125361, #88958 ) ;
#16034=FACE_OUTER_BOUND ( 'NONE', #102411, .T. ) ;
#16035=VERTEX_POINT ( 'NONE', #69311 ) ;
#16036=CIRCLE ( 'NONE', #120617, 0.06509327318403745899 ) ;
#16037=DIRECTION ( 'NONE',  ( 0.000000000000000000, 0.000000000000000000, -1.000000000000000000 ) ) ;
#16038=VERTEX_POINT ( 'NONE', #127609 ) ;
#16039=VERTEX_POINT ( 'NONE', #8455 ) ;
#16040=DIRECTION ( 'NONE',  ( -0.9974916312695812914, -0.05217691604166998370, 0.04783319955355741504 ) ) ;
#16041=VERTEX_POINT ( 'NONE', #77850 ) ;
#16042=DIRECTION ( 'NONE',  ( 0.000000000000000000, -0.000000000000000000, 1.000000000000000000 ) ) ;
#16043=DIRECTION ( 'NONE',  ( 0.000000000000000000, -0.000000000000000000, 1.000000000000000000 ) ) ;
#16044=AXIS2_PLACEMENT_3D ( 'NONE', #93640, #23603, #2022 ) ;
#16045=CIRCLE ( 'NONE', #91285, 0.06509327318403745899 ) ;
#16046=CARTESIAN_POINT ( 'NONE',  ( 5.849999999999933920, 12.50000000000000000, 6.495190528383297135 ) ) ;
#16047=VERTEX_POINT ( 'NONE', #59546 ) ;
#16048=VECTOR ( 'NONE', #36250, 1000.000000000000000 ) ;
#16049=FACE_BOUND ( 'NONE', #43371, .T. ) ;
#16050=CARTESIAN_POINT ( 'NONE',  ( 4.149999999999941735, 2.500000000000000000, -2.957883832488653830 ) ) ;
#16051=ORIENTED_EDGE ( 'NONE', *, *, #123893, .F. ) ;
#16052=CARTESIAN_POINT ( 'NONE',  ( -7.300000000000014921, 2.500000000000000000, 4.776537180435972196 ) ) ;
#16054=EDGE_LOOP ( 'NONE', ( #120403, #113981, #7982, #40861 ) ) ;
#16055=ORIENTED_EDGE ( 'NONE', *, *, #44379, .T. ) ;
#16056=ORIENTED_EDGE ( 'NONE', *, *, #46150, .F. ) ;
#16057=CARTESIAN_POINT ( 'NONE',  ( -11.89999999999999680, 2.500000000000000000, -0.2464101615137742063 ) ) ;
#16058=DIRECTION ( 'NONE',  ( 0.000000000000000000, 0.000000000000000000, 1.000000000000000000 ) ) ;
#16059=DIRECTION ( 'NONE',  ( -4.274815082592931898E-19, -0.9999939076577903929, -0.003490651415223739937 ) ) ;
#16060=FACE_BOUND ( 'NONE', #74229, .T. ) ;
#16061=VERTEX_POINT ( 'NONE', #128928 ) ;
#16062=AXIS2_PLACEMENT_3D ( 'NONE', #5011, #37077, #46234 ) ;
#16064=AXIS2_PLACEMENT_3D ( 'NONE', #29, #109994, #110630 ) ;
#16065=DIRECTION ( 'NONE',  ( 0.000000000000000000, 0.000000000000000000, 1.000000000000000000 ) ) ;
#16066=FACE_OUTER_BOUND ( 'NONE', #120, .T. ) ;
#16067=EDGE_CURVE ( 'NONE', #69354, #53159, #106037, .T. ) ;
#16068=LINE ( 'NONE', #26563, #103407 ) ;
#16069=AXIS2_PLACEMENT_3D ( 'NONE', #85929, #56474, #36219 ) ;
#16070=DIRECTION ( 'NONE',  ( 0.000000000000000000, 0.000000000000000000, 1.000000000000000000 ) ) ;
#16071=CARTESIAN_POINT ( 'NONE',  ( 12.69999999999990337, 12.50000000000000000, -4.676537180435978769 ) ) ;
#16072=CARTESIAN_POINT ( 'NONE',  ( 13.74999999999989875, 2.500000000000000000, 1.472243186433545459 ) ) ;
#16073=AXIS2_PLACEMENT_3D ( 'NONE', #17382, #48159, #57332 ) ;
#16074=DIRECTION ( 'NONE',  ( 0.000000000000000000, -0.9999939076577903929, 0.003490651415223739937 ) ) ;
#16075=DIRECTION ( 'NONE',  ( 0.000000000000000000, 0.000000000000000000, -1.000000000000000000 ) ) ;
#16076=CIRCLE ( 'NONE', #32848, 0.1000000000000000056 ) ;
#16077=ORIENTED_EDGE ( 'NONE', *, *, #31131, .T. ) ;
#16078=ORIENTED_EDGE ( 'NONE', *, *, #61721, .F. ) ;
#16079=VERTEX_POINT ( 'NONE', #99451 ) ;
#16080=ORIENTED_EDGE ( 'NONE', *, *, #9212, .T. ) ;
#16081=ORIENTED_EDGE ( 'NONE', *, *, #58613, .T. ) ;
#16082=DIRECTION ( 'NONE',  ( 0.000000000000000000, 0.000000000000000000, 1.000000000000000000 ) ) ;
#16083=DIRECTION ( 'NONE',  ( -0.000000000000000000, 1.000000000000000000, -0.000000000000000000 ) ) ;
#16084=VERTEX_POINT ( 'NONE', #108607 ) ;
#16085=FACE_BOUND ( 'NONE', #66446, .T. ) ;
#16086=CONICAL_SURFACE ( 'NONE', #9574, 0.1000000000000002554, 0.003490658503988666988 ) ;
#16087=CARTESIAN_POINT ( 'NONE',  ( -11.25000000000000178, 2.500000000000000000, -5.902370205355746968 ) ) ;
#16088=CONICAL_SURFACE ( 'NONE', #53678, 0.1000000000000002554, 0.003490658503988666988 ) ;
#16089=CONICAL_SURFACE ( 'NONE', #53679, 0.1000000000000002554, 0.003490658503988666988 ) ;
#16090=CARTESIAN_POINT ( 'NONE',  ( 1.899999999999951283, 2.500000000000000000, -0.2464101615137782308 ) ) ;
#16091=DIRECTION ( 'NONE',  ( 0.000000000000000000, -0.9999939076577903929, 0.003490651415223739937 ) ) ;
#16092=DIRECTION ( 'NONE',  ( 0.000000000000000000, 0.000000000000000000, 1.000000000000000000 ) ) ;
#16093=CARTESIAN_POINT ( 'NONE',  ( -5.200000000000022382, 2.500000000000000000, 4.776537180435972196 ) ) ;
#16094=VERTEX_POINT ( 'NONE', #100710 ) ;
#16095=CARTESIAN_POINT ( 'NONE',  ( -0.8500000000000395017, 2.500000000000000000, 2.165063509461097713 ) ) ;
#16096=VERTEX_POINT ( 'NONE', #28122 ) ;
#16097=ORIENTED_EDGE ( 'NONE', *, *, #18388, .F. ) ;
#16098=ORIENTED_EDGE ( 'NONE', *, *, #3017, .F. ) ;
#16099=DIRECTION ( 'NONE',  ( 0.000000000000000000, 0.000000000000000000, 1.000000000000000000 ) ) ;
#16100=LINE ( 'NONE', #95977, #127932 ) ;
#16101=CARTESIAN_POINT ( 'NONE',  ( -8.750000000000012434, 12.50000000000000000, -5.802370205355744659 ) ) ;
#16102=VERTEX_POINT ( 'NONE', #79792 ) ;
#16103=CONICAL_SURFACE ( 'NONE', #45389, 0.09999999999999982514, 0.003490658503988666988 ) ;
#16104=DIRECTION ( 'NONE',  ( 0.000000000000000000, 0.000000000000000000, -1.000000000000000000 ) ) ;
#16105=ADVANCED_FACE ( 'NONE', ( #88305 ), #32902, .T. ) ;
#16106=CARTESIAN_POINT ( 'NONE',  ( -10.00000000000000533, 2.500000000000000000, 0.6928203230275494784 ) ) ;
#16107=LINE ( 'NONE', #86138, #122703 ) ;
#16109=DIRECTION ( 'NONE',  ( 0.000000000000000000, -0.000000000000000000, 1.000000000000000000 ) ) ;
#16110=ADVANCED_FACE ( 'NONE', ( #70619 ), #70448, .T. ) ;
#16111=DIRECTION ( 'NONE',  ( 0.000000000000000000, -0.000000000000000000, 1.000000000000000000 ) ) ;
#16112=EDGE_CURVE ( 'NONE', #84287, #112495, #20365, .T. ) ;
#16113=ORIENTED_EDGE ( 'NONE', *, *, #57729, .F. ) ;
#16114=DIRECTION ( 'NONE',  ( 0.000000000000000000, 0.000000000000000000, -1.000000000000000000 ) ) ;
#16115=VERTEX_POINT ( 'NONE', #49712 ) ;
#16117=ORIENTED_EDGE ( 'NONE', *, *, #124308, .F. ) ;
#16118=DIRECTION ( 'NONE',  ( 0.000000000000000000, 0.000000000000000000, 1.000000000000000000 ) ) ;
#16119=EDGE_CURVE ( 'NONE', #80507, #59940, #57928, .T. ) ;
#16120=EDGE_CURVE ( 'NONE', #23223, #16380, #39258, .T. ) ;
#16121=CARTESIAN_POINT ( 'NONE',  ( 3.349999999999943689, 12.50000000000000000, 1.472243186433545459 ) ) ;
#16122=DIRECTION ( 'NONE',  ( -4.274815082592931898E-19, -0.9999939076577903929, -0.003490651415223739937 ) ) ;
#16123=EDGE_CURVE ( 'NONE', #1020, #12077, #99783, .T. ) ;
#16124=ORIENTED_EDGE ( 'NONE', *, *, #120664, .T. ) ;
#16125=AXIS2_PLACEMENT_3D ( 'NONE', #24122, #114420, #4441 ) ;
#16126=AXIS2_PLACEMENT_3D ( 'NONE', #2730, #61011, #121226 ) ;
#16129=DIRECTION ( 'NONE',  ( 0.000000000000000000, 0.000000000000000000, -1.000000000000000000 ) ) ;
#16130=DIRECTION ( 'NONE',  ( 0.000000000000000000, 0.000000000000000000, 1.000000000000000000 ) ) ;
#16131=VERTEX_POINT ( 'NONE', #118425 ) ;
#16132=ORIENTED_EDGE ( 'NONE', *, *, #73588, .T. ) ;
#16133=FACE_OUTER_BOUND ( 'NONE', #76544, .T. ) ;
#16134=CIRCLE ( 'NONE', #129057, 0.06509327318403745899 ) ;
#16135=CONICAL_SURFACE ( 'NONE', #74646, 0.1000000000000002554, 0.003490658503988666988 ) ;
#16136=VERTEX_POINT ( 'NONE', #129573 ) ;
#16137=DIRECTION ( 'NONE',  ( 0.000000000000000000, 0.000000000000000000, 1.000000000000000000 ) ) ;
#16138=AXIS2_PLACEMENT_3D ( 'NONE', #88550, #39488, #16572 ) ;
#16139=CARTESIAN_POINT ( 'NONE',  ( 3.949999999999938005, 2.500000000000000000, 6.741600689897071952 ) ) ;
#16140=EDGE_LOOP ( 'NONE', ( #75934, #39401, #77897, #51167 ) ) ;
#16141=FACE_OUTER_BOUND ( 'NONE', #40512, .T. ) ;
#16142=DIRECTION ( 'NONE',  ( 0.000000000000000000, 1.000000000000000000, 0.000000000000000000 ) ) ;
#16143=DIRECTION ( 'NONE',  ( 0.000000000000000000, 0.000000000000000000, 1.000000000000000000 ) ) ;
#16144=CARTESIAN_POINT ( 'NONE',  ( 10.59999999999991260, 12.50000000000000000, 0.4115034346978109769 ) ) ;
#16145=ORIENTED_EDGE ( 'NONE', *, *, #75659, .T. ) ;
#16146=DIRECTION ( 'NONE',  ( 0.000000000000000000, -0.9999939076577903929, 0.003490651415223739937 ) ) ;
#16147=AXIS2_PLACEMENT_3D ( 'NONE', #94107, #122698, #63129 ) ;
#16148=DIRECTION ( 'NONE',  ( 0.000000000000000000, 0.000000000000000000, 1.000000000000000000 ) ) ;
#16149=VERTEX_POINT ( 'NONE', #30066 ) ;
#16150=ORIENTED_EDGE ( 'NONE', *, *, #22020, .F. ) ;
#16152=DIRECTION ( 'NONE',  ( -0.000000000000000000, -1.000000000000000000, -0.000000000000000000 ) ) ;
#16153=DIRECTION ( 'NONE',  ( -0.000000000000000000, 1.000000000000000000, -0.000000000000000000 ) ) ;
#16154=DIRECTION ( 'NONE',  ( 0.000000000000000000, -0.9999939076577903929, 0.003490651415223739937 ) ) ;
#16155=CONICAL_SURFACE ( 'NONE', #45441, 0.1000000000000000472, 0.003490658503988666988 ) ;
#16156=DIRECTION ( 'NONE',  ( 0.000000000000000000, 1.000000000000000000, 0.000000000000000000 ) ) ;
#16157=AXIS2_PLACEMENT_3D ( 'NONE', #47631, #90105, #109102 ) ;
#16158=FACE_OUTER_BOUND ( 'NONE', #1531, .T. ) ;
#16159=AXIS2_PLACEMENT_3D ( 'NONE', #57925, #106994, #97828 ) ;
#16160=CARTESIAN_POINT ( 'NONE',  ( 17.50000000000000000, -2.500000000000000000, 0.000000000000000000 ) ) ;
#16161=DIRECTION ( 'NONE',  ( 0.000000000000000000, 1.000000000000000000, 0.000000000000000000 ) ) ;
#16162=CARTESIAN_POINT ( 'NONE',  ( 3.349999999999945466, 2.500000000000000000, -2.757883832488654097 ) ) ;
#16163=EDGE_CURVE ( 'NONE', #17352, #104853, #49066, .T. ) ;
#16164=EDGE_CURVE ( 'NONE', #11168, #93212, #9895, .T. ) ;
#16165=AXIS2_PLACEMENT_3D ( 'NONE', #119458, #19994, #39015 ) ;
#16166=EDGE_CURVE ( 'NONE', #868, #58932, #76797, .T. ) ;
#16167=FACE_OUTER_BOUND ( 'NONE', #104090, .T. ) ;
#16168=ORIENTED_EDGE ( 'NONE', *, *, #37887, .F. ) ;
#16170=AXIS2_PLACEMENT_3D ( 'NONE', #2676, #47140, #47782 ) ;
#16171=ORIENTED_EDGE ( 'NONE', *, *, #79246, .F. ) ;
#16172=FACE_OUTER_BOUND ( 'NONE', #45985, .T. ) ;
#16173=EDGE_CURVE ( 'NONE', #90210, #81351, #83068, .T. ) ;
#16174=EDGE_LOOP ( 'NONE', ( #30310, #71322 ) ) ;
#16175=AXIS2_PLACEMENT_3D ( 'NONE', #57531, #39840, #88246 ) ;
#16176=EDGE_CURVE ( 'NONE', #96180, #77015, #109240, .T. ) ;
#16177=PLANE ( 'NONE',  #125299 ) ;
#16178=CARTESIAN_POINT ( 'NONE',  ( -8.100000000000010303, 2.500000000000000000, 4.676537180435972552 ) ) ;
#16179=DIRECTION ( 'NONE',  ( 0.000000000000000000, 0.000000000000000000, -1.000000000000000000 ) ) ;
#16180=EDGE_CURVE ( 'NONE', #88083, #4728, #50998, .T. ) ;
#16181=VERTEX_POINT ( 'NONE', #83036 ) ;
#16182=EDGE_CURVE ( 'NONE', #118365, #94166, #26618, .T. ) ;
#16183=DIRECTION ( 'NONE',  ( 0.000000000000000000, 0.000000000000000000, 1.000000000000000000 ) ) ;
#16184=VECTOR ( 'NONE', #54000, 1000.000000000000000 ) ;
#16185=CONICAL_SURFACE ( 'NONE', #43318, 0.1000000000000002554, 0.003490658503988666988 ) ;
#16186=EDGE_CURVE ( 'NONE', #22692, #19600, #113774, .T. ) ;
#16187=DIRECTION ( 'NONE',  ( 0.000000000000000000, -0.9999939076577903929, 0.003490651415223739937 ) ) ;
#16188=ORIENTED_EDGE ( 'NONE', *, *, #61739, .T. ) ;
#16190=EDGE_CURVE ( 'NONE', #45761, #29933, #110155, .T. ) ;
#16191=DIRECTION ( 'NONE',  ( 0.000000000000000000, 0.000000000000000000, -1.000000000000000000 ) ) ;
#16192=ORIENTED_EDGE ( 'NONE', *, *, #90792, .T. ) ;
#16193=ORIENTED_EDGE ( 'NONE', *, *, #8881, .F. ) ;
#16194=ORIENTED_EDGE ( 'NONE', *, *, #38037, .T. ) ;
#16195=ORIENTED_EDGE ( 'NONE', *, *, #80922, .F. ) ;
#16196=CARTESIAN_POINT ( 'NONE',  ( 9.349999999999916156, 2.500000000000000000, -1.718653347947326049 ) ) ;
#16197=VECTOR ( 'NONE', #46033, 1000.000000000000000 ) ;
#16198=CARTESIAN_POINT ( 'NONE',  ( 4.799999999999934097, 2.500000000000000000, 4.676537180435972552 ) ) ;
#16199=DIRECTION ( 'NONE',  ( 0.000000000000000000, 0.000000000000000000, 1.000000000000000000 ) ) ;
#16200=DIRECTION ( 'NONE',  ( 0.000000000000000000, 0.000000000000000000, 1.000000000000000000 ) ) ;
#16202=CARTESIAN_POINT ( 'NONE',  ( 1.849999999999950573, 2.500000000000000000, 2.411473670974873862 ) ) ;
#16203=ORIENTED_EDGE ( 'NONE', *, *, #53619, .F. ) ;
#16204=CARTESIAN_POINT ( 'NONE',  ( -11.04999999999999893, 12.50000000000000000, 1.753560074763284016 ) ) ;
#16205=CARTESIAN_POINT ( 'NONE',  ( 15.83209681635555022, -2.499999999999998668, -5.404881881984142211 ) ) ;
#16206=DIRECTION ( 'NONE',  ( -1.000000000000000000, 0.000000000000000000, 0.000000000000000000 ) ) ;
#16207=CARTESIAN_POINT ( 'NONE',  ( 19.08853762629153294, -0.5565172524004106114, 4.470057054643206129 ) ) ;
#16208=ORIENTED_EDGE ( 'NONE', *, *, #83305, .F. ) ;
#16209=CIRCLE ( 'NONE', #35041, 0.06509327318403745899 ) ;
#16210=CIRCLE ( 'NONE', #122757, 0.06509327318403745899 ) ;
#16211=EDGE_LOOP ( 'NONE', ( #51531, #65778, #89267, #114530 ) ) ;
#16212=ORIENTED_EDGE ( 'NONE', *, *, #6761, .F. ) ;
#16213=DIRECTION ( 'NONE',  ( 0.000000000000000000, 0.000000000000000000, 1.000000000000000000 ) ) ;
#16214=DIRECTION ( 'NONE',  ( -0.000000000000000000, 1.000000000000000000, -0.000000000000000000 ) ) ;
#16215=CARTESIAN_POINT ( 'NONE',  ( -3.750000000000026201, 2.500000000000000000, 5.802370205355744659 ) ) ;
#16216=FACE_BOUND ( 'NONE', #46063, .T. ) ;
#16217=DIRECTION ( 'NONE',  ( 0.000000000000000000, -0.9999939076577903929, 0.003490651415223739937 ) ) ;
#16218=CARTESIAN_POINT ( 'NONE',  ( 2.699999999999945555, 12.50000000000000000, 3.983716857408420076 ) ) ;
#16219=AXIS2_PLACEMENT_3D ( 'NONE', #57876, #116132, #8112 ) ;
#16220=FACE_OUTER_BOUND ( 'NONE', #62689, .T. ) ;
#16221=DIRECTION ( 'NONE',  ( 0.000000000000000000, -0.000000000000000000, 1.000000000000000000 ) ) ;
#16222=AXIS2_PLACEMENT_3D ( 'NONE', #36781, #66855, #108072 ) ;
#16223=EDGE_CURVE ( 'NONE', #24379, #80231, #11943, .T. ) ;
#16224=AXIS2_PLACEMENT_3D ( 'NONE', #37964, #89651, #98164 ) ;
#16226=FACE_OUTER_BOUND ( 'NONE', #89756, .T. ) ;
#16227=PLANE ( 'NONE',  #107589 ) ;
#16228=CONICAL_SURFACE ( 'NONE', #26722, 0.1000000000000002554, 0.003490658503988666988 ) ;
#16229=DIRECTION ( 'NONE',  ( 0.000000000000000000, 0.000000000000000000, 1.000000000000000000 ) ) ;
#16230=ORIENTED_EDGE ( 'NONE', *, *, #14597, .F. ) ;
#16231=ORIENTED_EDGE ( 'NONE', *, *, #86683, .F. ) ;
#16232=VERTEX_POINT ( 'NONE', #62747 ) ;
#16233=ORIENTED_EDGE ( 'NONE', *, *, #92540, .F. ) ;
#16234=AXIS2_PLACEMENT_3D ( 'NONE', #127284, #29092, #59853 ) ;
#16236=CARTESIAN_POINT ( 'NONE',  ( -13.94999999999998863, 12.50000000000000000, -1.753560074763286458 ) ) ;
#16237=FACE_BOUND ( 'NONE', #65695, .T. ) ;
#16238=CARTESIAN_POINT ( 'NONE',  ( 10.84999999999991260, 2.500000000000000000, -2.165063509461101710 ) ) ;
#16239=AXIS2_PLACEMENT_3D ( 'NONE', #70176, #80646, #42000 ) ;
#16240=CIRCLE ( 'NONE', #43389, 0.06509327318403745899 ) ;
#16241=ORIENTED_EDGE ( 'NONE', *, *, #121972, .F. ) ;
#16242=DIRECTION ( 'NONE',  ( 0.000000000000000000, 1.000000000000000000, 0.000000000000000000 ) ) ;
#16243=DIRECTION ( 'NONE',  ( 0.000000000000000000, 0.000000000000000000, 1.000000000000000000 ) ) ;
#16244=AXIS2_PLACEMENT_3D ( 'NONE', #116416, #75849, #16272 ) ;
#16245=ORIENTED_EDGE ( 'NONE', *, *, #22980, .F. ) ;
#16246=DIRECTION ( 'NONE',  ( 0.000000000000000000, 0.000000000000000000, 1.000000000000000000 ) ) ;
#16247=CONICAL_SURFACE ( 'NONE', #28902, 0.1000000000000002554, 0.003490658503988666988 ) ;
#16248=DIRECTION ( 'NONE',  ( 0.000000000000000000, 0.000000000000000000, 1.000000000000000000 ) ) ;
#16249=AXIS2_PLACEMENT_3D ( 'NONE', #264, #30414, #50670 ) ;
#16250=ORIENTED_EDGE ( 'NONE', *, *, #6157, .F. ) ;
#16251=CARTESIAN_POINT ( 'NONE',  ( -2.900000000000030553, 12.50000000000000000, 5.022947341949748790 ) ) ;
#16252=DIRECTION ( 'NONE',  ( -4.274815082592931898E-19, -0.9999939076577903929, -0.003490651415223739937 ) ) ;
#16253=AXIS2_PLACEMENT_3D ( 'NONE', #114020, #122554, #21777 ) ;
#16254=AXIS2_PLACEMENT_3D ( 'NONE', #2937, #31749, #63132 ) ;
#16255=ORIENTED_EDGE ( 'NONE', *, *, #114771, .T. ) ;
#16256=CONICAL_SURFACE ( 'NONE', #47600, 0.09999999999999982514, 0.003490658503988666988 ) ;
#16257=EDGE_CURVE ( 'NONE', #114814, #78481, #118552, .T. ) ;
#16258=CARTESIAN_POINT ( 'NONE',  ( 4.599999999999937472, 2.500000000000000000, 0.6928203230275494784 ) ) ;
#16259=CARTESIAN_POINT ( 'NONE',  ( 9.599999999999914380, 12.50000000000000000, 4.265033745738159077 ) ) ;
#16260=ORIENTED_EDGE ( 'NONE', *, *, #122033, .F. ) ;
#16261=CARTESIAN_POINT ( 'NONE',  ( -8.350000000000008527, 2.500000000000000000, 5.902370205355745192 ) ) ;
#16262=ORIENTED_EDGE ( 'NONE', *, *, #90837, .T. ) ;
#16263=ORIENTED_EDGE ( 'NONE', *, *, #9374, .T. ) ;
#16264=CARTESIAN_POINT ( 'NONE',  ( -6.650000000000018119, 2.500000000000000000, -2.857883832488653741 ) ) ;
#16265=EDGE_CURVE ( 'NONE', #34182, #89915, #85100, .T. ) ;
#16267=CARTESIAN_POINT ( 'NONE',  ( 9.999999999999914735, 2.500000000000000000, 0.5928203230275495006 ) ) ;
#16268=FACE_BOUND ( 'NONE', #76097, .T. ) ;
#16269=CIRCLE ( 'NONE', #9944, 0.06509327318403743123 ) ;
#16270=CIRCLE ( 'NONE', #87300, 0.1000000000000002554 ) ;
#16271=ORIENTED_EDGE ( 'NONE', *, *, #35531, .F. ) ;
#16272=DIRECTION ( 'NONE',  ( 0.000000000000000000, 0.000000000000000000, -1.000000000000000000 ) ) ;
#16273=CARTESIAN_POINT ( 'NONE',  ( 10.59999999999990905, 2.500000000000000000, -4.576537180435978236 ) ) ;
#16274=DIRECTION ( 'NONE',  ( -0.000000000000000000, -1.000000000000000000, -0.000000000000000000 ) ) ;
#16275=EDGE_CURVE ( 'NONE', #69623, #73823, #78868, .T. ) ;
#16277=CARTESIAN_POINT ( 'NONE',  ( -0.4000000000000396572, 2.500000000000000000, 3.537306695894645081 ) ) ;
#16278=EDGE_CURVE ( 'NONE', #68489, #37844, #63381, .T. ) ;
#16279=FACE_OUTER_BOUND ( 'NONE', #77365, .T. ) ;
#16280=EDGE_CURVE ( 'NONE', #12101, #111595, #24099, .T. ) ;
#16281=EDGE_CURVE ( 'NONE', #47378, #102405, #108083, .T. ) ;
#16282=FACE_OUTER_BOUND ( 'NONE', #82879, .T. ) ;
#16284=ORIENTED_EDGE ( 'NONE', *, *, #51067, .T. ) ;
#16285=DIRECTION ( 'NONE',  ( 0.000000000000000000, 1.000000000000000000, 0.000000000000000000 ) ) ;
#16287=DIRECTION ( 'NONE',  ( -0.000000000000000000, -1.000000000000000000, -0.000000000000000000 ) ) ;
#16288=ORIENTED_EDGE ( 'NONE', *, *, #115585, .T. ) ;
#16289=ORIENTED_EDGE ( 'NONE', *, *, #51288, .F. ) ;
#16290=ORIENTED_EDGE ( 'NONE', *, *, #36152, .F. ) ;
#16291=ADVANCED_FACE ( 'NONE', ( #41189 ), #3811, .T. ) ;
#16292=DIRECTION ( 'NONE',  ( 0.000000000000000000, 0.000000000000000000, -1.000000000000000000 ) ) ;
#16293=DIRECTION ( 'NONE',  ( 0.000000000000000000, 0.000000000000000000, -1.000000000000000000 ) ) ;
#16294=EDGE_CURVE ( 'NONE', #85026, #98404, #45410, .T. ) ;
#16295=CARTESIAN_POINT ( 'NONE',  ( -13.14999999999999147, 2.500000000000000000, -1.818653347947323917 ) ) ;
#16297=DIRECTION ( 'NONE',  ( 0.000000000000000000, 0.000000000000000000, -1.000000000000000000 ) ) ;
#16298=CARTESIAN_POINT ( 'NONE',  ( 8.099999999999921485, 2.500000000000000000, -0.3464101615137783474 ) ) ;
#16299=DIRECTION ( 'NONE',  ( 0.000000000000000000, -0.000000000000000000, 1.000000000000000000 ) ) ;
#16300=CARTESIAN_POINT ( 'NONE',  ( -5.850000000000021849, 2.500000000000000000, -5.802370205355749988 ) ) ;
#16301=DIRECTION ( 'NONE',  ( 0.000000000000000000, 1.000000000000000000, 0.000000000000000000 ) ) ;
#16303=LINE ( 'NONE', #67996, #33262 ) ;
#16304=CIRCLE ( 'NONE', #43538, 0.1000000000000002554 ) ;
#16305=EDGE_LOOP ( 'NONE', ( #58859, #82297 ) ) ;
#16306=CIRCLE ( 'NONE', #79039, 0.1000000000000002554 ) ;
#16307=CARTESIAN_POINT ( 'NONE',  ( 2.099999999999950351, 2.500000000000000000, -4.330127018922201643 ) ) ;
#16308=ORIENTED_EDGE ( 'NONE', *, *, #125876, .T. ) ;
#16309=ORIENTED_EDGE ( 'NONE', *, *, #108668, .F. ) ;
#16310=CARTESIAN_POINT ( 'NONE',  ( -7.300000000000014921, 12.50000000000000000, 4.676537180435972552 ) ) ;
#16311=CARTESIAN_POINT ( 'NONE',  ( -10.85000000000000142, 2.500000000000000000, -1.472243186433546125 ) ) ;
#16312=DIRECTION ( 'NONE',  ( 0.000000000000000000, 1.000000000000000000, 0.000000000000000000 ) ) ;
#16313=DIRECTION ( 'NONE',  ( 0.000000000000000000, 1.000000000000000000, 0.000000000000000000 ) ) ;
#16314=AXIS2_PLACEMENT_3D ( 'NONE', #9794, #90267, #127633 ) ;
#16315=LINE ( 'NONE', #46434, #53168 ) ;
#16316=CARTESIAN_POINT ( 'NONE',  ( -5.850000000000018296, 2.500000000000000000, 1.472243186433545459 ) ) ;
#16317=EDGE_LOOP ( 'NONE', ( #103915, #98011, #21148, #25835 ) ) ;
#16318=DIRECTION ( 'NONE',  ( -0.000000000000000000, -1.000000000000000000, -0.000000000000000000 ) ) ;
#16319=ADVANCED_FACE ( 'NONE', ( #101376 ), #97714, .T. ) ;
#16320=DIRECTION ( 'NONE',  ( -4.274815082592931898E-19, -0.9999939076577903929, -0.003490651415223739937 ) ) ;
#16321=ORIENTED_EDGE ( 'NONE', *, *, #81897, .F. ) ;
#16322=AXIS2_PLACEMENT_3D ( 'NONE', #24819, #52994, #102714 ) ;
#16323=ORIENTED_EDGE ( 'NONE', *, *, #94092, .T. ) ;
#16324=EDGE_CURVE ( 'NONE', #65666, #103825, #70527, .T. ) ;
#16325=EDGE_LOOP ( 'NONE', ( #85807, #111209, #31255, #6898 ) ) ;
#16326=CIRCLE ( 'NONE', #12227, 0.06509327318403741736 ) ;
#16327=EDGE_CURVE ( 'NONE', #116425, #89261, #72568, .T. ) ;
#16329=DIRECTION ( 'NONE',  ( 0.000000000000000000, 1.000000000000000000, 0.000000000000000000 ) ) ;
#16330=CARTESIAN_POINT ( 'NONE',  ( -8.350000000000012079, 12.50000000000000000, 1.407149913249508000 ) ) ;
#16331=EDGE_CURVE ( 'NONE', #56423, #59088, #12334, .T. ) ;
#16332=CIRCLE ( 'NONE', #89516, 0.06509327318403745899 ) ;
#16333=DIRECTION ( 'NONE',  ( 0.000000000000000000, -0.9999939076577903929, 0.003490651415223739937 ) ) ;
#16334=DIRECTION ( 'NONE',  ( 0.000000000000000000, 0.000000000000000000, 1.000000000000000000 ) ) ;
#16335=EDGE_CURVE ( 'NONE', #111617, #75922, #84301, .T. ) ;
#16336=FACE_OUTER_BOUND ( 'NONE', #96187, .T. ) ;
#16337=EDGE_LOOP ( 'NONE', ( #9326, #34903 ) ) ;
#16338=DIRECTION ( 'NONE',  ( 0.000000000000000000, 1.000000000000000000, 0.000000000000000000 ) ) ;
#16339=AXIS2_PLACEMENT_3D ( 'NONE', #100989, #38887, #100358 ) ;
#16340=VECTOR ( 'NONE', #86333, 1000.000000000000000 ) ;
#16341=EDGE_CURVE ( 'NONE', #19741, #54151, #74743, .T. ) ;
#16342=CARTESIAN_POINT ( 'NONE',  ( 13.09999999999989839, 12.50000000000000000, 0.4115034346978109769 ) ) ;
#16343=ORIENTED_EDGE ( 'NONE', *, *, #9236, .T. ) ;
#16344=VECTOR ( 'NONE', #12511, 1000.000000000000000 ) ;
#16345=EDGE_LOOP ( 'NONE', ( #41643, #112515 ) ) ;
#16346=EDGE_LOOP ( 'NONE', ( #28624, #97760, #97602, #62414 ) ) ;
#16347=CARTESIAN_POINT ( 'NONE',  ( -7.900000000000011013, 2.500000000000000000, 3.637306695894644726 ) ) ;
#16348=CARTESIAN_POINT ( 'NONE',  ( -8.750000000000008882, 12.50000000000000000, 1.407149913249508000 ) ) ;
#16349=ORIENTED_EDGE ( 'NONE', *, *, #8051, .F. ) ;
#16350=DIRECTION ( 'NONE',  ( -0.000000000000000000, -1.000000000000000000, -0.000000000000000000 ) ) ;
#16351=LINE ( 'NONE', #56293, #51709 ) ;
#16353=DIRECTION ( 'NONE',  ( -0.000000000000000000, 1.000000000000000000, -0.000000000000000000 ) ) ;
#16354=CARTESIAN_POINT ( 'NONE',  ( -9.150000000000005684, 2.500000000000000000, 7.188010851410848723 ) ) ;
#16355=EDGE_CURVE ( 'NONE', #82690, #71646, #25365, .T. ) ;
#16356=CARTESIAN_POINT ( 'NONE',  ( -9.400000000000007461, 12.50000000000000000, 4.741630453620009789 ) ) ;
#16357=ORIENTED_EDGE ( 'NONE', *, *, #28169, .T. ) ;
#16358=AXIS2_PLACEMENT_3D ( 'NONE', #107449, #98265, #26964 ) ;
#16359=AXIS2_PLACEMENT_3D ( 'NONE', #74502, #122962, #24763 ) ;
#16360=FACE_OUTER_BOUND ( 'NONE', #50189, .T. ) ;
#16361=ORIENTED_EDGE ( 'NONE', *, *, #96035, .F. ) ;
#16362=ORIENTED_EDGE ( 'NONE', *, *, #74662, .T. ) ;
#16363=EDGE_LOOP ( 'NONE', ( #4866, #6904, #106559, #118151 ) ) ;
#16364=DIRECTION ( 'NONE',  ( 0.000000000000000000, 1.000000000000000000, 0.000000000000000000 ) ) ;
#16365=FACE_BOUND ( 'NONE', #123643, .T. ) ;
#16366=DIRECTION ( 'NONE',  ( 0.000000000000000000, 1.000000000000000000, 0.000000000000000000 ) ) ;
#16367=DIRECTION ( 'NONE',  ( 0.000000000000000000, 0.000000000000000000, -1.000000000000000000 ) ) ;
#16368=CARTESIAN_POINT ( 'NONE',  ( 0.7999999999999548583, 2.500000000000000000, 4.330127018922196314 ) ) ;
#16369=EDGE_CURVE ( 'NONE', #28068, #90204, #114436, .T. ) ;
#16370=CIRCLE ( 'NONE', #64510, 0.06509327318403745899 ) ;
#16371=ORIENTED_EDGE ( 'NONE', *, *, #108457, .F. ) ;
#16372=DIRECTION ( 'NONE',  ( 0.000000000000000000, 0.000000000000000000, -1.000000000000000000 ) ) ;
#16373=DIRECTION ( 'NONE',  ( 0.000000000000000000, 0.000000000000000000, 1.000000000000000000 ) ) ;
#16374=LINE ( 'NONE', #25561, #59113 ) ;
#16375=DIRECTION ( 'NONE',  ( -0.000000000000000000, 1.000000000000000000, -0.000000000000000000 ) ) ;
#16376=ORIENTED_EDGE ( 'NONE', *, *, #82253, .F. ) ;
#16378=CARTESIAN_POINT ( 'NONE',  ( 12.49999999999990585, 2.500000000000000000, -5.022947341949754119 ) ) ;
#16379=VECTOR ( 'NONE', #16776, 1000.000000000000000 ) ;
#16380=VERTEX_POINT ( 'NONE', #16817 ) ;
#16381=DIRECTION ( 'NONE',  ( 0.000000000000000000, 1.000000000000000000, 0.000000000000000000 ) ) ;
#16382=ADVANCED_FACE ( 'NONE', ( #5087 ), #58024, .T. ) ;
#16383=FACE_BOUND ( 'NONE', #57436, .T. ) ;
#16384=DIRECTION ( 'NONE',  ( 0.000000000000000000, 0.000000000000000000, 1.000000000000000000 ) ) ;
#16385=CIRCLE ( 'NONE', #108353, 0.06509327318403745899 ) ;
#16386=CIRCLE ( 'NONE', #26885, 0.09999999999999982514 ) ;
#16387=AXIS2_PLACEMENT_3D ( 'NONE', #75939, #54371, #85117 ) ;
#16388=VERTEX_POINT ( 'NONE', #94766 ) ;
#16390=CARTESIAN_POINT ( 'NONE',  ( -11.84999999999999787, 2.500000000000000000, -6.841600689897074261 ) ) ;
#16391=EDGE_LOOP ( 'NONE', ( #38360, #33158, #58479, #24184 ) ) ;
#16392=ORIENTED_EDGE ( 'NONE', *, *, #72633, .F. ) ;
#16394=CONICAL_SURFACE ( 'NONE', #89595, 0.1000000000000000472, 0.003490658503988666988 ) ;
#16395=ORIENTED_EDGE ( 'NONE', *, *, #82551, .T. ) ;
#16397=DIRECTION ( 'NONE',  ( -0.000000000000000000, -1.000000000000000000, -0.000000000000000000 ) ) ;
#16398=DIRECTION ( 'NONE',  ( 0.000000000000000000, 0.000000000000000000, -1.000000000000000000 ) ) ;
#16399=DIRECTION ( 'NONE',  ( -0.000000000000000000, 1.000000000000000000, -0.000000000000000000 ) ) ;
#16400=DIRECTION ( 'NONE',  ( -0.000000000000000000, -1.000000000000000000, -0.000000000000000000 ) ) ;
#16401=CIRCLE ( 'NONE', #45790, 0.1000000000000002554 ) ;
#16402=EDGE_LOOP ( 'NONE', ( #20389, #124595 ) ) ;
#16403=EDGE_CURVE ( 'NONE', #40177, #67175, #120705, .T. ) ;
#16404=CARTESIAN_POINT ( 'NONE',  ( 4.149999999999938183, 2.500000000000000000, 5.802370205355744659 ) ) ;
#16405=CARTESIAN_POINT ( 'NONE',  ( 6.649999999999930189, 12.50000000000000000, 7.188010851410848723 ) ) ;
#16406=AXIS2_PLACEMENT_3D ( 'NONE', #108843, #19162, #36907 ) ;
#16407=DIRECTION ( 'NONE',  ( 0.000000000000000000, 1.000000000000000000, 0.000000000000000000 ) ) ;
#16408=DIRECTION ( 'NONE',  ( 0.000000000000000000, 1.000000000000000000, 0.000000000000000000 ) ) ;
#16409=ORIENTED_EDGE ( 'NONE', *, *, #8631, .T. ) ;
#16410=ORIENTED_EDGE ( 'NONE', *, *, #64843, .T. ) ;
#16411=FACE_BOUND ( 'NONE', #9562, .T. ) ;
#16412=VERTEX_POINT ( 'NONE', #94124 ) ;
#16413=DIRECTION ( 'NONE',  ( -0.000000000000000000, -1.000000000000000000, -0.000000000000000000 ) ) ;
#16414=LINE ( 'NONE', #74725, #22751 ) ;
#16415=ORIENTED_EDGE ( 'NONE', *, *, #25968, .T. ) ;
#16416=DIRECTION ( 'NONE',  ( 0.000000000000000000, 1.000000000000000000, 0.000000000000000000 ) ) ;
#16417=EDGE_CURVE ( 'NONE', #12263, #48527, #18294, .T. ) ;
#16418=AXIS2_PLACEMENT_3D ( 'NONE', #43746, #115015, #94743 ) ;
#16419=CARTESIAN_POINT ( 'NONE',  ( 5.399999999999934630, 12.50000000000000000, -0.6277270498435167934 ) ) ;
#16420=CARTESIAN_POINT ( 'NONE',  ( 11.24999999999994493, 12.50000000000000000, -2.165063509461101710 ) ) ;
#16421=CARTESIAN_POINT ( 'NONE',  ( -0.6000000000000388356, 2.500000000000000000, 3.883716857408421319 ) ) ;
#16422=VERTEX_POINT ( 'NONE', #96052 ) ;
#16424=CARTESIAN_POINT ( 'NONE',  ( 9.349999999999919709, 2.500000000000000000, -6.841600689897078702 ) ) ;
#16425=LINE ( 'NONE', #57008, #16680 ) ;
#16426=EDGE_CURVE ( 'NONE', #128319, #41444, #30845, .T. ) ;
#16427=EDGE_CURVE ( 'NONE', #79210, #16232, #64266, .T. ) ;
#16428=CARTESIAN_POINT ( 'NONE',  ( 0.3999999999999563904, 2.500000000000000000, 5.122947341949749323 ) ) ;
#16430=EDGE_CURVE ( 'NONE', #120997, #4440, #36514, .T. ) ;
#16431=ADVANCED_FACE ( 'NONE', ( #45042 ), #76425, .T. ) ;
#16432=AXIS2_PLACEMENT_3D ( 'NONE', #57873, #108246, #55288 ) ;
#16434=CONICAL_SURFACE ( 'NONE', #14388, 0.1000000000000002554, 0.003490658503988666988 ) ;
#16435=EDGE_LOOP ( 'NONE', ( #95201, #103654 ) ) ;
#16436=ORIENTED_EDGE ( 'NONE', *, *, #21618, .T. ) ;
#16437=DIRECTION ( 'NONE',  ( 0.000000000000000000, 1.000000000000000000, 0.000000000000000000 ) ) ;
#16438=EDGE_CURVE ( 'NONE', #87504, #19669, #98183, .T. ) ;
#16440=ADVANCED_FACE ( 'NONE', ( #116968 ), #115037, .T. ) ;
#16441=DIRECTION ( 'NONE',  ( 0.000000000000000000, -0.000000000000000000, 1.000000000000000000 ) ) ;
#16442=ORIENTED_EDGE ( 'NONE', *, *, #27611, .T. ) ;
#16443=VERTEX_POINT ( 'NONE', #6355 ) ;
#16444=EDGE_LOOP ( 'NONE', ( #77980, #19718 ) ) ;
#16445=CONICAL_SURFACE ( 'NONE', #85420, 0.09999999999999982514, 0.003490658503988666988 ) ;
#16446=EDGE_CURVE ( 'NONE', #126127, #68087, #46302, .T. ) ;
#16447=CARTESIAN_POINT ( 'NONE',  ( 2.099999999999949463, 2.500000000000000000, 0.5928203230275495006 ) ) ;
#16448=ADVANCED_FACE ( 'NONE', ( #95418 ), #10450, .T. ) ;
#16449=DIRECTION ( 'NONE',  ( 0.000000000000000000, 0.000000000000000000, -1.000000000000000000 ) ) ;
#16450=EDGE_CURVE ( 'NONE', #14174, #57147, #94081, .T. ) ;
#16451=DIRECTION ( 'NONE',  ( 0.000000000000000000, 1.000000000000000000, 0.000000000000000000 ) ) ;
#16453=AXIS2_PLACEMENT_3D ( 'NONE', #119875, #129081, #20392 ) ;
#16454=AXIS2_PLACEMENT_3D ( 'NONE', #124274, #83706, #92890 ) ;
#16455=CARTESIAN_POINT ( 'NONE',  ( -0.6500000000000403233, 2.500000000000000000, 1.818653347947321475 ) ) ;
#16456=DIRECTION ( 'NONE',  ( 0.000000000000000000, 0.000000000000000000, -1.000000000000000000 ) ) ;
#16457=CARTESIAN_POINT ( 'NONE',  ( 13.74999999999989519, 2.500000000000000000, -2.957883832488653830 ) ) ;
#16458=CIRCLE ( 'NONE', #1789, 0.06509327318403741736 ) ;
#16459=EDGE_LOOP ( 'NONE', ( #70195, #121954, #13772, #77318 ) ) ;
#16460=EDGE_CURVE ( 'NONE', #6759, #14824, #125510, .T. ) ;
#16461=FACE_OUTER_BOUND ( 'NONE', #64567, .T. ) ;
#16462=EDGE_LOOP ( 'NONE', ( #21789, #62752, #87963, #105308 ) ) ;
#16463=CIRCLE ( 'NONE', #81239, 0.1000000000000002554 ) ;
#16464=AXIS2_PLACEMENT_3D ( 'NONE', #124891, #62759, #115047 ) ;
#16465=ORIENTED_EDGE ( 'NONE', *, *, #55031, .T. ) ;
#16466=ORIENTED_EDGE ( 'NONE', *, *, #30221, .T. ) ;
#16467=EDGE_LOOP ( 'NONE', ( #120300, #68805 ) ) ;
#16468=PLANE ( 'NONE',  #102829 ) ;
#16470=VERTEX_POINT ( 'NONE', #32193 ) ;
#16471=DIRECTION ( 'NONE',  ( -0.000000000000000000, -1.000000000000000000, -0.000000000000000000 ) ) ;
#16472=FACE_OUTER_BOUND ( 'NONE', #29634, .T. ) ;
#16473=CARTESIAN_POINT ( 'NONE',  ( -1.900000000000034994, 12.50000000000000000, -0.3464101615137783474 ) ) ;
#16474=CARTESIAN_POINT ( 'NONE',  ( -4.150000000000025224, 2.500000000000000000, 7.188010851410848723 ) ) ;
#16475=CARTESIAN_POINT ( 'NONE',  ( 12.09999999999990550, 2.500000000000000000, 4.430127018922196847 ) ) ;
#16476=AXIS2_PLACEMENT_3D ( 'NONE', #2927, #3560, #128840 ) ;
#16477=ORIENTED_EDGE ( 'NONE', *, *, #85736, .T. ) ;
#16478=FACE_OUTER_BOUND ( 'NONE', #78538, .T. ) ;
#16479=ORIENTED_EDGE ( 'NONE', *, *, #95772, .T. ) ;
#16480=CONICAL_SURFACE ( 'NONE', #83412, 0.09999999999999999167, 0.003490658503988666988 ) ;
#16481=DIRECTION ( 'NONE',  ( 0.000000000000000000, 1.000000000000000000, 0.000000000000000000 ) ) ;
#16482=CIRCLE ( 'NONE', #29042, 0.1000000000000002554 ) ;
#16483=ORIENTED_EDGE ( 'NONE', *, *, #93932, .T. ) ;
#16484=DIRECTION ( 'NONE',  ( -0.000000000000000000, 1.000000000000000000, -0.000000000000000000 ) ) ;
#16485=VERTEX_POINT ( 'NONE', #44568 ) ;
#16486=ORIENTED_EDGE ( 'NONE', *, *, #80592, .T. ) ;
#16487=DIRECTION ( 'NONE',  ( 0.000000000000000000, 0.000000000000000000, -1.000000000000000000 ) ) ;
#16488=CIRCLE ( 'NONE', #81375, 0.1000000000000002554 ) ;
#16489=FACE_OUTER_BOUND ( 'NONE', #57641, .T. ) ;
#16490=CONICAL_SURFACE ( 'NONE', #110595, 0.1000000000000002554, 0.003490658503988666988 ) ;
#16491=ADVANCED_FACE ( 'NONE', ( #51821 ), #62698, .T. ) ;
#16492=AXIS2_PLACEMENT_3D ( 'NONE', #7619, #47569, #28567 ) ;
#16494=FACE_OUTER_BOUND ( 'NONE', #13130, .T. ) ;
#16495=EDGE_CURVE ( 'NONE', #100499, #76783, #121174, .T. ) ;
#16496=CARTESIAN_POINT ( 'NONE',  ( -7.950000000000012612, 2.500000000000000000, -2.065063509461102065 ) ) ;
#16497=ORIENTED_EDGE ( 'NONE', *, *, #120806, .T. ) ;
#16498=FACE_OUTER_BOUND ( 'NONE', #4929, .T. ) ;
#16499=DIRECTION ( 'NONE',  ( 0.000000000000000000, 0.000000000000000000, -1.000000000000000000 ) ) ;
#16500=DIRECTION ( 'NONE',  ( 0.000000000000000000, -0.9999939076577903929, 0.003490651415223739937 ) ) ;
#16501=DIRECTION ( 'NONE',  ( 0.000000000000000000, 1.000000000000000000, 0.000000000000000000 ) ) ;
#16502=AXIS2_PLACEMENT_3D ( 'NONE', #53447, #115548, #44911 ) ;
#16503=ADVANCED_FACE ( 'NONE', ( #94295 ), #60648, .T. ) ;
#16504=DIRECTION ( 'NONE',  ( -0.000000000000000000, -1.000000000000000000, -0.000000000000000000 ) ) ;
#16505=AXIS2_PLACEMENT_3D ( 'NONE', #121637, #121002, #81088 ) ;
#16506=ORIENTED_EDGE ( 'NONE', *, *, #3445, .T. ) ;
#16507=ORIENTED_EDGE ( 'NONE', *, *, #22412, .F. ) ;
#16508=CARTESIAN_POINT ( 'NONE',  ( 5.849999999999932143, 12.50000000000000000, 2.165063509461097713 ) ) ;
#16509=VERTEX_POINT ( 'NONE', #72743 ) ;
#16510=CARTESIAN_POINT ( 'NONE',  ( 12.69999999999990337, 12.50000000000000000, -4.741630453620016006 ) ) ;
#16511=DIRECTION ( 'NONE',  ( 0.000000000000000000, -0.000000000000000000, 1.000000000000000000 ) ) ;
#16512=CIRCLE ( 'NONE', #93613, 0.06509327318403745899 ) ;
#16513=CIRCLE ( 'NONE', #27007, 0.09999999999999982514 ) ;
#16514=ORIENTED_EDGE ( 'NONE', *, *, #84758, .T. ) ;
#16516=DIRECTION ( 'NONE',  ( 0.000000000000000000, 0.000000000000000000, 1.000000000000000000 ) ) ;
#16517=DIRECTION ( 'NONE',  ( -0.000000000000000000, -1.000000000000000000, -0.000000000000000000 ) ) ;
#16518=CARTESIAN_POINT ( 'NONE',  ( -1.900000000000035438, 2.500000000000000000, 3.883716857408420431 ) ) ;
#16520=EDGE_LOOP ( 'NONE', ( #51444, #69183, #81002, #20250 ) ) ;
#16521=DIRECTION ( 'NONE',  ( 0.000000000000000000, 0.000000000000000000, 1.000000000000000000 ) ) ;
#16522=LINE ( 'NONE', #74181, #93647 ) ;
#16523=VECTOR ( 'NONE', #65762, 1000.000000000000000 ) ;
#16524=ORIENTED_EDGE ( 'NONE', *, *, #7482, .T. ) ;
#16525=DIRECTION ( 'NONE',  ( 0.000000000000000000, 0.000000000000000000, 1.000000000000000000 ) ) ;
#16526=CARTESIAN_POINT ( 'NONE',  ( 6.249999999999934275, 2.500000000000000000, -7.188010851410854052 ) ) ;
#16527=DIRECTION ( 'NONE',  ( 0.000000000000000000, 0.000000000000000000, 1.000000000000000000 ) ) ;
#16528=VECTOR ( 'NONE', #5586, 1000.000000000000000 ) ;
#16529=VERTEX_POINT ( 'NONE', #121827 ) ;
#16530=CARTESIAN_POINT ( 'NONE',  ( -3.750000000000026201, 12.50000000000000000, 5.867463478539781896 ) ) ;
#16531=VERTEX_POINT ( 'NONE', #11868 ) ;
#16532=DIRECTION ( 'NONE',  ( 0.000000000000000000, 1.000000000000000000, 0.000000000000000000 ) ) ;
#16533=VECTOR ( 'NONE', #65063, 1000.000000000000000 ) ;
#16534=FACE_OUTER_BOUND ( 'NONE', #44425, .T. ) ;
#16535=CARTESIAN_POINT ( 'NONE',  ( 5.199999999999931788, 12.50000000000000000, 4.676537180435972552 ) ) ;
#16536=ORIENTED_EDGE ( 'NONE', *, *, #4412, .F. ) ;
#16537=DIRECTION ( 'NONE',  ( 0.000000000000000000, 0.000000000000000000, 1.000000000000000000 ) ) ;
#16538=CIRCLE ( 'NONE', #125322, 0.1000000000000002554 ) ;
#16539=AXIS2_PLACEMENT_3D ( 'NONE', #86256, #18172, #97381 ) ;
#16540=CARTESIAN_POINT ( 'NONE',  ( 11.64999999999990798, 12.50000000000000000, -2.857883832488653741 ) ) ;
#16542=CIRCLE ( 'NONE', #20778, 0.06509327318403745899 ) ;
#16543=VERTEX_POINT ( 'NONE', #52443 ) ;
#16545=EDGE_LOOP ( 'NONE', ( #95098, #29187, #61582, #6561 ) ) ;
#16546=DIRECTION ( 'NONE',  ( 0.000000000000000000, 0.000000000000000000, 1.000000000000000000 ) ) ;
#16547=AXIS2_PLACEMENT_3D ( 'NONE', #113752, #54184, #124852 ) ;
#16548=CONICAL_SURFACE ( 'NONE', #125240, 0.1000000000000002554, 0.003490658503988666988 ) ;
#16549=VERTEX_POINT ( 'NONE', #111347 ) ;
#16550=DIRECTION ( 'NONE',  ( 0.000000000000000000, 0.000000000000000000, 1.000000000000000000 ) ) ;
#16551=CARTESIAN_POINT ( 'NONE',  ( 6.049999999999932321, 2.500000000000000000, -1.818653347947326138 ) ) ;
#16552=ORIENTED_EDGE ( 'NONE', *, *, #105207, .T. ) ;
#16553=EDGE_CURVE ( 'NONE', #122658, #31101, #102207, .T. ) ;
#16554=ORIENTED_EDGE ( 'NONE', *, *, #30060, .T. ) ;
#16555=CARTESIAN_POINT ( 'NONE',  ( 7.899999999999924860, 2.500000000000000000, -5.022947341949754119 ) ) ;
#16556=CARTESIAN_POINT ( 'NONE',  ( -3.300000000000027800, 2.500000000000000000, -0.1000000000000022815 ) ) ;
#16558=DIRECTION ( 'NONE',  ( 0.000000000000000000, 1.000000000000000000, 0.000000000000000000 ) ) ;
#16560=PLANE ( 'NONE',  #7496 ) ;
#16561=CONICAL_SURFACE ( 'NONE', #45839, 0.1000000000000000472, 0.003490658503988666988 ) ;
#16563=DIRECTION ( 'NONE',  ( 0.000000000000000000, -0.000000000000000000, 1.000000000000000000 ) ) ;
#16565=AXIS2_PLACEMENT_3D ( 'NONE', #2502, #11698, #100713 ) ;
#16566=CIRCLE ( 'NONE', #39610, 0.06509327318403741736 ) ;
#16567=ORIENTED_EDGE ( 'NONE', *, *, #111498, .T. ) ;
#16569=ORIENTED_EDGE ( 'NONE', *, *, #29039, .T. ) ;
#16570=ORIENTED_EDGE ( 'NONE', *, *, #28964, .T. ) ;
#16571=ORIENTED_EDGE ( 'NONE', *, *, #116165, .T. ) ;
#16572=DIRECTION ( 'NONE',  ( 0.000000000000000000, 0.000000000000000000, 1.000000000000000000 ) ) ;
#16573=DIRECTION ( 'NONE',  ( -0.000000000000000000, 1.000000000000000000, -0.000000000000000000 ) ) ;
#16574=CARTESIAN_POINT ( 'NONE',  ( 10.64999999999991331, 2.500000000000000000, -2.611473670974877592 ) ) ;
#16575=VERTEX_POINT ( 'NONE', #123130 ) ;
#16576=FACE_BOUND ( 'NONE', #32379, .T. ) ;
#16577=DIRECTION ( 'NONE',  ( -0.000000000000000000, 1.000000000000000000, -0.000000000000000000 ) ) ;
#16578=LINE ( 'NONE', #127215, #66811 ) ;
#16579=AXIS2_PLACEMENT_3D ( 'NONE', #53876, #43434, #93806 ) ;
#16580=CIRCLE ( 'NONE', #29141, 0.06509327318403745899 ) ;
#16581=DIRECTION ( 'NONE',  ( 0.000000000000000000, 0.000000000000000000, 1.000000000000000000 ) ) ;
#16582=EDGE_CURVE ( 'NONE', #50154, #72001, #82572, .T. ) ;
#16583=CONICAL_SURFACE ( 'NONE', #81378, 0.1000000000000000472, 0.003490658503988666988 ) ;
#16584=CARTESIAN_POINT ( 'NONE',  ( 3.549999999999943867, 12.50000000000000000, -6.148780366869526226 ) ) ;
#16585=DIRECTION ( 'NONE',  ( 0.000000000000000000, 1.000000000000000000, 0.000000000000000000 ) ) ;
#16586=CARTESIAN_POINT ( 'NONE',  ( 3.749999999999942268, 2.500000000000000000, 1.572243186433545548 ) ) ;
#16587=CARTESIAN_POINT ( 'NONE',  ( 14.79999999999989235, 2.500000000000000000, 0.4464101615137735513 ) ) ;
#16588=DIRECTION ( 'NONE',  ( 0.000000000000000000, -0.9999939076577903929, 0.003490651415223739937 ) ) ;
#16589=ADVANCED_FACE ( 'NONE', ( #21710 ), #106589, .T. ) ;
#16590=EDGE_CURVE ( 'NONE', #51103, #10534, #23632, .T. ) ;
#16591=DIRECTION ( 'NONE',  ( -0.000000000000000000, 1.000000000000000000, -0.000000000000000000 ) ) ;
#16592=EDGE_CURVE ( 'NONE', #46680, #68655, #101558, .T. ) ;
#16593=AXIS2_PLACEMENT_3D ( 'NONE', #31083, #122024, #41546 ) ;
#16595=CARTESIAN_POINT ( 'NONE',  ( 4.799999999999935874, 2.500000000000000000, 4.083716857408421497 ) ) ;
#16596=CIRCLE ( 'NONE', #56311, 0.1000000000000002554 ) ;
#16598=ORIENTED_EDGE ( 'NONE', *, *, #37486, .T. ) ;
#16599=VECTOR ( 'NONE', #121836, 1000.000000000000000 ) ;
#16600=EDGE_LOOP ( 'NONE', ( #35494, #50085 ) ) ;
#16601=EDGE_LOOP ( 'NONE', ( #97725, #47242 ) ) ;
#16602=DIRECTION ( 'NONE',  ( 0.000000000000000000, -0.000000000000000000, 1.000000000000000000 ) ) ;
#16603=EDGE_CURVE ( 'NONE', #101658, #55263, #43292, .T. ) ;
#16604=FACE_OUTER_BOUND ( 'NONE', #2201, .T. ) ;
#16606=ORIENTED_EDGE ( 'NONE', *, *, #32285, .T. ) ;
#16607=VERTEX_POINT ( 'NONE', #83831 ) ;
#16608=CARTESIAN_POINT ( 'NONE',  ( 2.499999999999945377, 2.500000000000000000, 5.022947341949748790 ) ) ;
#16609=EDGE_CURVE ( 'NONE', #85331, #86064, #123747, .T. ) ;
#16610=CARTESIAN_POINT ( 'NONE',  ( 2.899999999999946620, 2.500000000000000000, -3.637306695894650055 ) ) ;
#16611=CARTESIAN_POINT ( 'NONE',  ( -7.700000000000012612, 2.500000000000000000, 4.676537180435972552 ) ) ;
#16612=CARTESIAN_POINT ( 'NONE',  ( 11.89999999999990798, 2.500000000000000000, -4.776537180435977525 ) ) ;
#16613=AXIS2_PLACEMENT_3D ( 'NONE', #20503, #89233, #19177 ) ;
#16614=CARTESIAN_POINT ( 'NONE',  ( -2.300000000000033573, 2.500000000000000000, 4.576537180435972019 ) ) ;
#16615=EDGE_CURVE ( 'NONE', #91437, #111265, #89870, .T. ) ;
#16616=VERTEX_POINT ( 'NONE', #77249 ) ;
#16617=EDGE_CURVE ( 'NONE', #1046, #124254, #48115, .T. ) ;
#16618=ORIENTED_EDGE ( 'NONE', *, *, #58112, .T. ) ;
#16619=ORIENTED_EDGE ( 'NONE', *, *, #36442, .F. ) ;
#16620=ORIENTED_EDGE ( 'NONE', *, *, #118428, .T. ) ;
#16621=LINE ( 'NONE', #56551, #71386 ) ;
#16622=EDGE_LOOP ( 'NONE', ( #120775, #113843, #72183, #124320 ) ) ;
#16623=ORIENTED_EDGE ( 'NONE', *, *, #67788, .F. ) ;
#16624=LINE ( 'NONE', #56554, #128066 ) ;
#16625=DIRECTION ( 'NONE',  ( 0.000000000000000000, 0.000000000000000000, -1.000000000000000000 ) ) ;
#16626=CARTESIAN_POINT ( 'NONE',  ( -8.750000000000010658, 2.500000000000000000, -1.372243186433550033 ) ) ;
#16627=DIRECTION ( 'NONE',  ( 0.000000000000000000, 0.000000000000000000, 1.000000000000000000 ) ) ;
#16628=PLANE ( 'NONE',  #55950 ) ;
#16629=CIRCLE ( 'NONE', #54219, 0.06509327318403745899 ) ;
#16630=VERTEX_POINT ( 'NONE', #36696 ) ;
#16631=DIRECTION ( 'NONE',  ( 0.000000000000000000, 0.000000000000000000, 1.000000000000000000 ) ) ;
#16633=DIRECTION ( 'NONE',  ( 0.000000000000000000, 1.000000000000000000, 0.000000000000000000 ) ) ;
#16635=AXIS2_PLACEMENT_3D ( 'NONE', #10903, #129457, #69865 ) ;
#16636=ORIENTED_EDGE ( 'NONE', *, *, #125113, .T. ) ;
#16638=DIRECTION ( 'NONE',  ( 0.000000000000000000, 0.000000000000000000, 1.000000000000000000 ) ) ;
#16639=ORIENTED_EDGE ( 'NONE', *, *, #50196, .T. ) ;
#16640=VECTOR ( 'NONE', #27072, 1000.000000000000000 ) ;
#16641=DIRECTION ( 'NONE',  ( 0.000000000000000000, 1.000000000000000000, 0.000000000000000000 ) ) ;
#16642=LINE ( 'NONE', #46780, #96108 ) ;
#16643=ORIENTED_EDGE ( 'NONE', *, *, #57575, .T. ) ;
#16644=CIRCLE ( 'NONE', #41729, 0.06509327318403745899 ) ;
#16645=VECTOR ( 'NONE', #11875, 1000.000000000000000 ) ;
#16646=EDGE_CURVE ( 'NONE', #55594, #41939, #68945, .T. ) ;
#16647=DIRECTION ( 'NONE',  ( 0.000000000000000000, 0.000000000000000000, 1.000000000000000000 ) ) ;
#16648=EDGE_CURVE ( 'NONE', #100324, #116919, #58508, .T. ) ;
#16649=EDGE_LOOP ( 'NONE', ( #10638, #91892 ) ) ;
#16650=ORIENTED_EDGE ( 'NONE', *, *, #103920, .F. ) ;
#16652=DIRECTION ( 'NONE',  ( -0.000000000000000000, -1.000000000000000000, -0.000000000000000000 ) ) ;
#16654=CARTESIAN_POINT ( 'NONE',  ( -8.100000000000013856, 2.500000000000000000, -4.083716857408426826 ) ) ;
#16655=FACE_OUTER_BOUND ( 'NONE', #70257, .T. ) ;
#16656=DIRECTION ( 'NONE',  ( 0.000000000000000000, 0.000000000000000000, 1.000000000000000000 ) ) ;
#16657=ORIENTED_EDGE ( 'NONE', *, *, #44132, .T. ) ;
#16658=LINE ( 'NONE', #87338, #50692 ) ;
#16659=CONICAL_SURFACE ( 'NONE', #8354, 0.09999999999999982514, 0.003490658503988666988 ) ;
#16660=CONICAL_SURFACE ( 'NONE', #2005, 0.1000000000000000472, 0.003490658503988666988 ) ;
#16661=EDGE_LOOP ( 'NONE', ( #90317, #84106, #126959, #20929 ) ) ;
#16662=DIRECTION ( 'NONE',  ( 0.000000000000000000, 0.000000000000000000, 1.000000000000000000 ) ) ;
#16663=CARTESIAN_POINT ( 'NONE',  ( 6.449999999999928235, 2.500000000000000000, 2.611473670974873151 ) ) ;
#16664=DIRECTION ( 'NONE',  ( -0.000000000000000000, -1.000000000000000000, -0.000000000000000000 ) ) ;
#16665=CARTESIAN_POINT ( 'NONE',  ( 13.29999999999990301, 2.500000000000000000, -4.230127018922201998 ) ) ;
#16666=ORIENTED_EDGE ( 'NONE', *, *, #82999, .F. ) ;
#16667=CIRCLE ( 'NONE', #112842, 0.06509327318403745899 ) ;
#16668=VECTOR ( 'NONE', #76046, 1000.000000000000000 ) ;
#16669=DIRECTION ( 'NONE',  ( -0.000000000000000000, 1.000000000000000000, -0.000000000000000000 ) ) ;
#16670=DIRECTION ( 'NONE',  ( -0.000000000000000000, 1.000000000000000000, -0.000000000000000000 ) ) ;
#16671=AXIS2_PLACEMENT_3D ( 'NONE', #94989, #5296, #75331 ) ;
#16672=ORIENTED_EDGE ( 'NONE', *, *, #76784, .T. ) ;
#16673=DIRECTION ( 'NONE',  ( 0.000000000000000000, 0.000000000000000000, -1.000000000000000000 ) ) ;
#16674=AXIS2_PLACEMENT_3D ( 'NONE', #117276, #125200, #75441 ) ;
#16675=ADVANCED_FACE ( 'NONE', ( #126999 ), #29253, .T. ) ;
#16676=AXIS2_PLACEMENT_3D ( 'NONE', #15742, #63577, #5910 ) ;
#16677=ORIENTED_EDGE ( 'NONE', *, *, #12461, .T. ) ;
#16678=ORIENTED_EDGE ( 'NONE', *, *, #113396, .T. ) ;
#16679=CARTESIAN_POINT ( 'NONE',  ( 13.09999999999989839, 2.500000000000000000, 0.4464101615137735513 ) ) ;
#16680=VECTOR ( 'NONE', #89069, 1000.000000000000000 ) ;
#16682=DIRECTION ( 'NONE',  ( 0.000000000000000000, 1.000000000000000000, 0.000000000000000000 ) ) ;
#16683=DIRECTION ( 'NONE',  ( -4.274815082592931898E-19, -0.9999939076577903929, -0.003490651415223739937 ) ) ;
#16685=CARTESIAN_POINT ( 'NONE',  ( -12.29999999999999361, 2.500000000000000000, 3.983716857408420076 ) ) ;
#16686=EDGE_CURVE ( 'NONE', #45115, #68393, #37656, .T. ) ;
#16687=VERTEX_POINT ( 'NONE', #126351 ) ;
#16688=FACE_BOUND ( 'NONE', #90500, .T. ) ;
#16689=CARTESIAN_POINT ( 'NONE',  ( -7.700000000000014388, 12.50000000000000000, -0.2813168883297408329 ) ) ;
#16690=VERTEX_POINT ( 'NONE', #37340 ) ;
#16691=AXIS2_PLACEMENT_3D ( 'NONE', #104768, #35419, #73389 ) ;
#16692=EDGE_CURVE ( 'NONE', #102068, #81635, #7849, .T. ) ;
#16693=CARTESIAN_POINT ( 'NONE',  ( 9.149999999999916866, 2.500000000000000000, 7.088010851410848190 ) ) ;
#16694=LINE ( 'NONE', #116197, #42580 ) ;
#16695=ADVANCED_FACE ( 'NONE', ( #87056 ), #25037, .T. ) ;
#16697=ORIENTED_EDGE ( 'NONE', *, *, #3181, .T. ) ;
#16698=ORIENTED_EDGE ( 'NONE', *, *, #8733, .F. ) ;
#16699=CARTESIAN_POINT ( 'NONE',  ( 14.59999999999989484, 12.50000000000000000, -0.6928203230275541413 ) ) ;
#16700=CARTESIAN_POINT ( 'NONE',  ( -6.249999999999984901, 2.500000000000000000, -2.265063509461101798 ) ) ;
#16701=DIRECTION ( 'NONE',  ( -0.000000000000000000, 1.000000000000000000, -0.000000000000000000 ) ) ;
#16702=EDGE_CURVE ( 'NONE', #120532, #80728, #54363, .T. ) ;
#16703=FACE_BOUND ( 'NONE', #29135, .T. ) ;
#16706=CARTESIAN_POINT ( 'NONE',  ( 9.349999999999919709, 12.50000000000000000, -6.148780366869526226 ) ) ;
#16707=CARTESIAN_POINT ( 'NONE',  ( -7.100000000000017408, 2.500000000000000000, -5.122947341949753763 ) ) ;
#16708=DIRECTION ( 'NONE',  ( -0.000000000000000000, -1.000000000000000000, -0.000000000000000000 ) ) ;
#16709=DIRECTION ( 'NONE',  ( 0.000000000000000000, 0.000000000000000000, 1.000000000000000000 ) ) ;
#16710=PLANE ( 'NONE',  #92537 ) ;
#16711=AXIS2_PLACEMENT_3D ( 'NONE', #115123, #96788, #35321 ) ;
#16712=PLANE ( 'NONE',  #3225 ) ;
#16713=DIRECTION ( 'NONE',  ( -0.000000000000000000, 1.000000000000000000, -0.000000000000000000 ) ) ;
#16714=VECTOR ( 'NONE', #86722, 1000.000000000000000 ) ;
#16715=CONICAL_SURFACE ( 'NONE', #2063, 0.1000000000000002554, 0.003490658503988666988 ) ;
#16716=ORIENTED_EDGE ( 'NONE', *, *, #62285, .T. ) ;
#16717=ORIENTED_EDGE ( 'NONE', *, *, #69111, .F. ) ;
#16718=VERTEX_POINT ( 'NONE', #116517 ) ;
#16719=ORIENTED_EDGE ( 'NONE', *, *, #27662, .F. ) ;
#16720=VERTEX_POINT ( 'NONE', #35397 ) ;
#16721=CARTESIAN_POINT ( 'NONE',  ( -10.00000000000000533, 12.50000000000000000, 5.088040615133786027 ) ) ;
#16722=CARTESIAN_POINT ( 'NONE',  ( 7.949999999999922018, 2.500000000000000000, -2.265063509461101798 ) ) ;
#16724=FACE_BOUND ( 'NONE', #77246, .T. ) ;
#16725=DIRECTION ( 'NONE',  ( 0.000000000000000000, 1.000000000000000000, 0.000000000000000000 ) ) ;
#16726=AXIS2_PLACEMENT_3D ( 'NONE', #57079, #85887, #36175 ) ;
#16727=AXIS2_PLACEMENT_3D ( 'NONE', #66773, #106698, #87062 ) ;
#16728=ADVANCED_FACE ( 'NONE', ( #96876 ), #47796, .T. ) ;
#16729=CARTESIAN_POINT ( 'NONE',  ( -2.100000000000033840, 2.500000000000000000, 3.737306695894644371 ) ) ;
#16730=CARTESIAN_POINT ( 'NONE',  ( 2.500000000000002220, -1.500000000000000000, 10.00000000000000178 ) ) ;
#16731=DIRECTION ( 'NONE',  ( 0.000000000000000000, 1.000000000000000000, 0.000000000000000000 ) ) ;
#16732=EDGE_CURVE ( 'NONE', #50402, #113932, #31400, .T. ) ;
#16733=LINE ( 'NONE', #16093, #83019 ) ;
#16734=ORIENTED_EDGE ( 'NONE', *, *, #57247, .F. ) ;
#16735=DIRECTION ( 'NONE',  ( 0.000000000000000000, 1.000000000000000000, 0.000000000000000000 ) ) ;
#16736=ADVANCED_FACE ( 'NONE', ( #87700 ), #75203, .T. ) ;
#16737=VERTEX_POINT ( 'NONE', #66769 ) ;
#16738=EDGE_LOOP ( 'NONE', ( #59294, #4799, #86621, #105705 ) ) ;
#16739=ORIENTED_EDGE ( 'NONE', *, *, #89317, .F. ) ;
#16740=EDGE_CURVE ( 'NONE', #10395, #2451, #2035, .T. ) ;
#16741=LINE ( 'NONE', #39025, #119559 ) ;
#16742=DIRECTION ( 'NONE',  ( 0.000000000000000000, -0.000000000000000000, 1.000000000000000000 ) ) ;
#16743=EDGE_CURVE ( 'NONE', #41301, #52849, #52230, .T. ) ;
#16744=DIRECTION ( 'NONE',  ( 0.000000000000000000, -0.000000000000000000, 1.000000000000000000 ) ) ;
#16745=EDGE_CURVE ( 'NONE', #84287, #53425, #95601, .T. ) ;
#16746=EDGE_LOOP ( 'NONE', ( #19005, #23209, #98715, #56108 ) ) ;
#16747=DIRECTION ( 'NONE',  ( 0.000000000000000000, 0.000000000000000000, -1.000000000000000000 ) ) ;
#16748=EDGE_CURVE ( 'NONE', #18481, #45029, #48199, .T. ) ;
#16749=AXIS2_PLACEMENT_3D ( 'NONE', #78487, #107921, #87626 ) ;
#16751=AXIS2_PLACEMENT_3D ( 'NONE', #118673, #88572, #78777 ) ;
#16752=CARTESIAN_POINT ( 'NONE',  ( 1.649999999999950617, 2.500000000000000000, 2.065063509461097624 ) ) ;
#16753=EDGE_CURVE ( 'NONE', #69211, #27373, #108738, .T. ) ;
#16755=DIRECTION ( 'NONE',  ( 0.000000000000000000, 0.000000000000000000, 1.000000000000000000 ) ) ;
#16756=DIRECTION ( 'NONE',  ( 0.000000000000000000, 1.000000000000000000, 0.000000000000000000 ) ) ;
#16757=CARTESIAN_POINT ( 'NONE',  ( 10.64999999999991331, 2.500000000000000000, 6.248780366869521430 ) ) ;
#16758=ORIENTED_EDGE ( 'NONE', *, *, #126734, .T. ) ;
#16759=CARTESIAN_POINT ( 'NONE',  ( -12.09999999999999609, 2.500000000000000000, 1.734723475976807094E-15 ) ) ;
#16760=ADVANCED_FACE ( 'NONE', ( #127634 ), #37965, .T. ) ;
#16761=EDGE_LOOP ( 'NONE', ( #111456, #11193 ) ) ;
#16762=ORIENTED_EDGE ( 'NONE', *, *, #65044, .F. ) ;
#16763=CARTESIAN_POINT ( 'NONE',  ( -6.050000000000018474, 2.500000000000000000, 2.511473670974873507 ) ) ;
#16764=CARTESIAN_POINT ( 'NONE',  ( -7.100000000000017408, 2.500000000000000000, -4.922947341949753586 ) ) ;
#16765=LINE ( 'NONE', #95363, #92705 ) ;
#16766=CIRCLE ( 'NONE', #33538, 0.06509327318403745899 ) ;
#16767=ORIENTED_EDGE ( 'NONE', *, *, #29954, .T. ) ;
#16768=EDGE_LOOP ( 'NONE', ( #111242, #28770, #32355, #102578 ) ) ;
#16769=CONICAL_SURFACE ( 'NONE', #27334, 0.09999999999999982514, 0.003490658503988666988 ) ;
#16771=CIRCLE ( 'NONE', #83708, 0.06509327318403745899 ) ;
#16772=CARTESIAN_POINT ( 'NONE',  ( -10.65000000000000391, 12.50000000000000000, -6.083687093685485436 ) ) ;
#16773=CARTESIAN_POINT ( 'NONE',  ( 15.39999999999989200, 12.50000000000000000, -0.6928203230275542523 ) ) ;
#16774=ORIENTED_EDGE ( 'NONE', *, *, #64312, .T. ) ;
#16775=ORIENTED_EDGE ( 'NONE', *, *, #93254, .T. ) ;
#16776=DIRECTION ( 'NONE',  ( -4.274815082592931898E-19, -0.9999939076577903929, -0.003490651415223739937 ) ) ;
#16777=AXIS2_PLACEMENT_3D ( 'NONE', #71282, #43155, #11727 ) ;
#16778=VERTEX_POINT ( 'NONE', #19621 ) ;
#16779=FACE_OUTER_BOUND ( 'NONE', #90509, .T. ) ;
#16780=DIRECTION ( 'NONE',  ( 0.000000000000000000, 0.000000000000000000, 1.000000000000000000 ) ) ;
#16781=VERTEX_POINT ( 'NONE', #9151 ) ;
#16782=CARTESIAN_POINT ( 'NONE',  ( 8.149999999999923972, 2.500000000000000000, 1.818653347947321475 ) ) ;
#16783=LINE ( 'NONE', #96636, #2390 ) ;
#16784=AXIS2_PLACEMENT_3D ( 'NONE', #93686, #4629, #43951 ) ;
#16785=DIRECTION ( 'NONE',  ( 0.000000000000000000, -0.000000000000000000, 1.000000000000000000 ) ) ;
#16786=DIRECTION ( 'NONE',  ( -0.000000000000000000, 1.000000000000000000, -0.000000000000000000 ) ) ;
#16787=VERTEX_POINT ( 'NONE', #18316 ) ;
#16788=DIRECTION ( 'NONE',  ( 0.000000000000000000, 0.000000000000000000, 1.000000000000000000 ) ) ;
#16789=EDGE_CURVE ( 'NONE', #122997, #79131, #29342, .T. ) ;
#16790=DIRECTION ( 'NONE',  ( -0.000000000000000000, -1.000000000000000000, -0.000000000000000000 ) ) ;
#16791=ORIENTED_EDGE ( 'NONE', *, *, #56745, .F. ) ;
#16792=EDGE_LOOP ( 'NONE', ( #96318, #64009 ) ) ;
#16793=FACE_OUTER_BOUND ( 'NONE', #115796, .T. ) ;
#16794=CARTESIAN_POINT ( 'NONE',  ( -11.44999999999999751, 2.500000000000000000, 6.741600689897071952 ) ) ;
#16795=CARTESIAN_POINT ( 'NONE',  ( -4.150000000000025224, 12.50000000000000000, 5.737276932171707422 ) ) ;
#16796=DIRECTION ( 'NONE',  ( 0.000000000000000000, 0.000000000000000000, -1.000000000000000000 ) ) ;
#16797=CARTESIAN_POINT ( 'NONE',  ( -7.900000000000014566, 12.50000000000000000, -0.6928203230275541413 ) ) ;
#16798=DIRECTION ( 'NONE',  ( -0.000000000000000000, -1.000000000000000000, -0.000000000000000000 ) ) ;
#16799=ADVANCED_FACE ( 'NONE', ( #88330 ), #52315, .T. ) ;
#16800=CARTESIAN_POINT ( 'NONE',  ( -6.650000000000018119, 12.50000000000000000, -2.857883832488653741 ) ) ;
#16801=DIRECTION ( 'NONE',  ( 0.000000000000000000, 0.000000000000000000, 1.000000000000000000 ) ) ;
#16802=CARTESIAN_POINT ( 'NONE',  ( 8.949999999999921130, 12.50000000000000000, -6.776507416713040577 ) ) ;
#16803=AXIS2_PLACEMENT_3D ( 'NONE', #2300, #2971, #21984 ) ;
#16804=AXIS2_PLACEMENT_3D ( 'NONE', #38400, #98557, #107099 ) ;
#16805=CARTESIAN_POINT ( 'NONE',  ( 13.74999999999993427, 12.50000000000000000, 2.165063509461097713 ) ) ;
#16806=ORIENTED_EDGE ( 'NONE', *, *, #40239, .T. ) ;
#16807=AXIS2_PLACEMENT_3D ( 'NONE', #80786, #20567, #121332 ) ;
#16808=ORIENTED_EDGE ( 'NONE', *, *, #91572, .T. ) ;
#16809=DIRECTION ( 'NONE',  ( 0.000000000000000000, 1.000000000000000000, 0.000000000000000000 ) ) ;
#16810=ORIENTED_EDGE ( 'NONE', *, *, #4734, .F. ) ;
#16811=LINE ( 'NONE', #54824, #91748 ) ;
#16812=DIRECTION ( 'NONE',  ( -0.000000000000000000, 1.000000000000000000, -0.000000000000000000 ) ) ;
#16814=ORIENTED_EDGE ( 'NONE', *, *, #95210, .F. ) ;
#16815=CARTESIAN_POINT ( 'NONE',  ( 19.01901804971413767, -2.576149587736929369, -2.431039412660861210 ) ) ;
#16816=CARTESIAN_POINT ( 'NONE',  ( 13.54999999999990123, 2.500000000000000000, 1.818653347947321475 ) ) ;
#16817=CARTESIAN_POINT ( 'NONE',  ( -2.500000000000032419, 2.500000000000000000, 0.5928203230275495006 ) ) ;
#16818=ORIENTED_EDGE ( 'NONE', *, *, #13017, .T. ) ;
#16819=DIRECTION ( 'NONE',  ( 0.000000000000000000, 1.000000000000000000, 0.000000000000000000 ) ) ;
#16820=ORIENTED_EDGE ( 'NONE', *, *, #127155, .F. ) ;
#16821=EDGE_CURVE ( 'NONE', #8340, #87068, #83716, .T. ) ;
#16822=ORIENTED_EDGE ( 'NONE', *, *, #96975, .F. ) ;
#16823=VERTEX_POINT ( 'NONE', #48431 ) ;
#16824=ORIENTED_EDGE ( 'NONE', *, *, #109684, .F. ) ;
#16825=CARTESIAN_POINT ( 'NONE',  ( 5.199999999999933564, 2.500000000000000000, 0.3464101615137735735 ) ) ;
#16826=CARTESIAN_POINT ( 'NONE',  ( -0.2000000000000412836, 2.500000000000000000, 4.676537180435972552 ) ) ;
#16828=DIRECTION ( 'NONE',  ( 0.000000000000000000, 1.000000000000000000, 0.000000000000000000 ) ) ;
#16829=EDGE_CURVE ( 'NONE', #71159, #79454, #9796, .T. ) ;
#16830=ORIENTED_EDGE ( 'NONE', *, *, #104618, .T. ) ;
#16831=CONICAL_SURFACE ( 'NONE', #60870, 0.1000000000000000056, 0.003490658503988666988 ) ;
#16832=DIRECTION ( 'NONE',  ( 0.000000000000000000, 0.000000000000000000, 1.000000000000000000 ) ) ;
#16833=VERTEX_POINT ( 'NONE', #10437 ) ;
#16834=LINE ( 'NONE', #115706, #30844 ) ;
#16835=DIRECTION ( 'NONE',  ( 0.000000000000000000, 1.000000000000000000, 0.000000000000000000 ) ) ;
#16836=ADVANCED_FACE ( 'NONE', ( #89009 ), #73244, .T. ) ;
#16837=CARTESIAN_POINT ( 'NONE',  ( 6.449999999999930012, 2.500000000000000000, -1.918653347947326004 ) ) ;
#16838=CARTESIAN_POINT ( 'NONE',  ( 19.72570408286438592, -0.6078483229322464432, 4.299616118078763094 ) ) ;
#16839=ADVANCED_FACE ( 'NONE', ( #58266 ), #60729, .T. ) ;
#16840=CIRCLE ( 'NONE', #35667, 0.09999999999999999167 ) ;
#16841=EDGE_LOOP ( 'NONE', ( #8665, #74626 ) ) ;
#16842=VERTEX_POINT ( 'NONE', #99481 ) ;
#16843=EDGE_CURVE ( 'NONE', #7520, #47255, #87885, .T. ) ;
#16844=ORIENTED_EDGE ( 'NONE', *, *, #128399, .F. ) ;
#16845=CARTESIAN_POINT ( 'NONE',  ( 7.299999999999927880, 2.500000000000000000, 3.983716857408420964 ) ) ;
#16846=PLANE ( 'NONE',  #72771 ) ;
#16847=FACE_OUTER_BOUND ( 'NONE', #94627, .T. ) ;
#16848=ADVANCED_FACE ( 'NONE', ( #40575 ), #10531, .T. ) ;
#16849=FACE_BOUND ( 'NONE', #12362, .T. ) ;
#16850=CARTESIAN_POINT ( 'NONE',  ( 0.1999999999999571565, 2.500000000000000000, 3.883716857408420431 ) ) ;
#16851=DIRECTION ( 'NONE',  ( 0.000000000000000000, 1.000000000000000000, 0.000000000000000000 ) ) ;
#16852=DIRECTION ( 'NONE',  ( 0.000000000000000000, 1.000000000000000000, 0.000000000000000000 ) ) ;
#16853=CARTESIAN_POINT ( 'NONE',  ( 7.299999999999927880, 12.50000000000000000, -4.676537180435977881 ) ) ;
#16854=AXIS2_PLACEMENT_3D ( 'NONE', #10420, #107977, #88316 ) ;
#16855=CONICAL_SURFACE ( 'NONE', #96297, 0.1000000000000000472, 0.003490658503988666988 ) ;
#16857=DIRECTION ( 'NONE',  ( -0.000000000000000000, 1.000000000000000000, -0.000000000000000000 ) ) ;
#16858=FACE_OUTER_BOUND ( 'NONE', #12386, .T. ) ;
#16859=AXIS2_PLACEMENT_3D ( 'NONE', #34618, #84337, #36548 ) ;
#16860=PLANE ( 'NONE',  #22250 ) ;
#16861=VERTEX_POINT ( 'NONE', #108635 ) ;
#16862=CONICAL_SURFACE ( 'NONE', #31486, 0.1000000000000002554, 0.003490658503988666988 ) ;
#16863=EDGE_LOOP ( 'NONE', ( #4234, #85534 ) ) ;
#16864=ORIENTED_EDGE ( 'NONE', *, *, #17592, .F. ) ;
#16865=ORIENTED_EDGE ( 'NONE', *, *, #49749, .F. ) ;
#16866=DIRECTION ( 'NONE',  ( -0.000000000000000000, -1.000000000000000000, -0.000000000000000000 ) ) ;
#16867=FACE_BOUND ( 'NONE', #76428, .T. ) ;
#16869=CARTESIAN_POINT ( 'NONE',  ( 6.449999999999930012, 2.500000000000000000, -1.918653347947326004 ) ) ;
#16870=ORIENTED_EDGE ( 'NONE', *, *, #650, .F. ) ;
#16871=LINE ( 'NONE', #46362, #46726 ) ;
#16873=ORIENTED_EDGE ( 'NONE', *, *, #26783, .T. ) ;
#16874=DIRECTION ( 'NONE',  ( 0.000000000000000000, 0.000000000000000000, 1.000000000000000000 ) ) ;
#16875=CARTESIAN_POINT ( 'NONE',  ( 17.79089025268845603, 2.511997385349134859, -2.795007471442833236 ) ) ;
#16876=AXIS2_PLACEMENT_3D ( 'NONE', #20361, #129049, #10522 ) ;
#16877=EDGE_CURVE ( 'NONE', #112226, #90933, #89957, .T. ) ;
#16878=ORIENTED_EDGE ( 'NONE', *, *, #94997, .T. ) ;
#16879=EDGE_CURVE ( 'NONE', #117157, #113704, #8472, .T. ) ;
#16880=FACE_OUTER_BOUND ( 'NONE', #112802, .T. ) ;
#16881=AXIS2_PLACEMENT_3D ( 'NONE', #113559, #63825, #123376 ) ;
#16882=CARTESIAN_POINT ( 'NONE',  ( -9.350000000000008527, 12.50000000000000000, -6.148780366869520897 ) ) ;
#16883=EDGE_CURVE ( 'NONE', #87020, #10181, #119213, .T. ) ;
#16884=EDGE_CURVE ( 'NONE', #118072, #40034, #69346, .T. ) ;
#16885=EDGE_LOOP ( 'NONE', ( #47450, #37963, #16308, #28231 ) ) ;
#16886=CARTESIAN_POINT ( 'NONE',  ( -5.600000000000023626, 2.500000000000000000, -3.983716857408426293 ) ) ;
#16887=AXIS2_PLACEMENT_3D ( 'NONE', #19769, #109434, #120542 ) ;
#16888=FACE_OUTER_BOUND ( 'NONE', #32024, .T. ) ;
#16889=VERTEX_POINT ( 'NONE', #120405 ) ;
#16890=CARTESIAN_POINT ( 'NONE',  ( 11.89999999999990798, 12.50000000000000000, 4.676537180435972552 ) ) ;
#16891=EDGE_CURVE ( 'NONE', #42074, #123090, #58586, .T. ) ;
#16892=ORIENTED_EDGE ( 'NONE', *, *, #92572, .F. ) ;
#16893=VECTOR ( 'NONE', #7609, 1000.000000000000000 ) ;
#16894=VERTEX_POINT ( 'NONE', #129599 ) ;
#16896=EDGE_LOOP ( 'NONE', ( #53111, #21230, #37831, #50850 ) ) ;
#16897=DIRECTION ( 'NONE',  ( -0.000000000000000000, -1.000000000000000000, -0.000000000000000000 ) ) ;
#16898=DIRECTION ( 'NONE',  ( 0.000000000000000000, 0.000000000000000000, 1.000000000000000000 ) ) ;
#16899=EDGE_CURVE ( 'NONE', #14536, #85204, #41864, .T. ) ;
#16900=EDGE_CURVE ( 'NONE', #49639, #106042, #100118, .T. ) ;
#16901=ORIENTED_EDGE ( 'NONE', *, *, #112977, .T. ) ;
#16902=DIRECTION ( 'NONE',  ( 0.000000000000000000, -0.000000000000000000, 1.000000000000000000 ) ) ;
#16903=ORIENTED_EDGE ( 'NONE', *, *, #106865, .F. ) ;
#16904=LINE ( 'NONE', #86310, #50396 ) ;
#16905=DIRECTION ( 'NONE',  ( 0.000000000000000000, 0.000000000000000000, 1.000000000000000000 ) ) ;
#16907=DIRECTION ( 'NONE',  ( -0.000000000000000000, -1.000000000000000000, -0.000000000000000000 ) ) ;
#16908=CARTESIAN_POINT ( 'NONE',  ( -9.600000000000008527, 2.500000000000000000, 4.430127018922196847 ) ) ;
#16909=ORIENTED_EDGE ( 'NONE', *, *, #8366, .T. ) ;
#16910=ORIENTED_EDGE ( 'NONE', *, *, #79140, .T. ) ;
#16911=CIRCLE ( 'NONE', #102623, 0.1000000000000000472 ) ;
#16912=DIRECTION ( 'NONE',  ( 0.000000000000000000, 0.000000000000000000, 1.000000000000000000 ) ) ;
#16913=CARTESIAN_POINT ( 'NONE',  ( 21.24754738303277080, -0.7337760880902354232, 4.182111650399362723 ) ) ;
#16914=CARTESIAN_POINT ( 'NONE',  ( -9.800000000000006040, 2.500000000000000000, 4.776537180435972196 ) ) ;
#16915=EDGE_LOOP ( 'NONE', ( #123598, #44146, #108798, #20319 ) ) ;
#16916=ORIENTED_EDGE ( 'NONE', *, *, #116798, .T. ) ;
#16917=ORIENTED_EDGE ( 'NONE', *, *, #50360, .F. ) ;
#16918=CARTESIAN_POINT ( 'NONE',  ( -1.850000000000033396, 2.500000000000000000, -2.411473670974877859 ) ) ;
#16919=VECTOR ( 'NONE', #41181, 1000.000000000000000 ) ;
#16920=CARTESIAN_POINT ( 'NONE',  ( 15.83209681635555377, 1.499999999999999556, 5.404881881984147540 ) ) ;
#16921=CONICAL_SURFACE ( 'NONE', #10676, 0.09999999999999982514, 0.003490658503988666988 ) ;
#16922=DIRECTION ( 'NONE',  ( 0.000000000000000000, -0.000000000000000000, 1.000000000000000000 ) ) ;
#16924=DIRECTION ( 'NONE',  ( -4.274815082592931898E-19, -0.9999939076577903929, -0.003490651415223739937 ) ) ;
#16926=DIRECTION ( 'NONE',  ( -0.000000000000000000, -1.000000000000000000, -0.000000000000000000 ) ) ;
#16928=DIRECTION ( 'NONE',  ( -4.274815082592931898E-19, -0.9999939076577903929, -0.003490651415223739937 ) ) ;
#16929=CARTESIAN_POINT ( 'NONE',  ( -6.450000000000019718, 12.50000000000000000, -1.883746621131363597 ) ) ;
#16930=CIRCLE ( 'NONE', #98431, 0.06509327318403745899 ) ;
#16931=CIRCLE ( 'NONE', #90108, 0.09999999999999982514 ) ;
#16934=ORIENTED_EDGE ( 'NONE', *, *, #11310, .T. ) ;
#16935=VERTEX_POINT ( 'NONE', #113807 ) ;
#16936=DIRECTION ( 'NONE',  ( 0.000000000000000000, 0.000000000000000000, -1.000000000000000000 ) ) ;
#16937=CARTESIAN_POINT ( 'NONE',  ( -6.700000000000016165, 2.500000000000000000, 4.430127018922196847 ) ) ;
#16938=CARTESIAN_POINT ( 'NONE',  ( -3.350000000000031619, 12.50000000000000000, -7.188010851410854052 ) ) ;
#16939=VECTOR ( 'NONE', #59397, 1000.000000000000000 ) ;
#16940=DIRECTION ( 'NONE',  ( 0.000000000000000000, -0.9999939076577903929, 0.003490651415223739937 ) ) ;
#16941=AXIS2_PLACEMENT_3D ( 'NONE', #66464, #99164, #38311 ) ;
#16942=EDGE_CURVE ( 'NONE', #56443, #126922, #14724, .T. ) ;
#16943=CARTESIAN_POINT ( 'NONE',  ( 4.149999999999941735, 12.50000000000000000, -7.188010851410854052 ) ) ;
#16944=FACE_OUTER_BOUND ( 'NONE', #112119, .T. ) ;
#16945=DIRECTION ( 'NONE',  ( -0.000000000000000000, -1.000000000000000000, -0.000000000000000000 ) ) ;
#16946=ORIENTED_EDGE ( 'NONE', *, *, #41474, .T. ) ;
#16947=DIRECTION ( 'NONE',  ( 0.000000000000000000, 1.000000000000000000, 0.000000000000000000 ) ) ;
#16948=AXIS2_PLACEMENT_3D ( 'NONE', #24624, #126691, #65817 ) ;
#16949=CARTESIAN_POINT ( 'NONE',  ( 0.7999999999999553024, 2.500000000000000000, -4.430127018922202176 ) ) ;
#16950=ORIENTED_EDGE ( 'NONE', *, *, #36108, .T. ) ;
#16951=ORIENTED_EDGE ( 'NONE', *, *, #67563, .T. ) ;
#16952=CIRCLE ( 'NONE', #21098, 0.1000000000000002554 ) ;
#16953=CIRCLE ( 'NONE', #85930, 0.1000000000000002554 ) ;
#16954=VERTEX_POINT ( 'NONE', #52303 ) ;
#16955=ORIENTED_EDGE ( 'NONE', *, *, #85529, .F. ) ;
#16956=ORIENTED_EDGE ( 'NONE', *, *, #14401, .T. ) ;
#16957=DIRECTION ( 'NONE',  ( 0.000000000000000000, 1.000000000000000000, 0.000000000000000000 ) ) ;
#16958=DIRECTION ( 'NONE',  ( 0.000000000000000000, 0.000000000000000000, 1.000000000000000000 ) ) ;
#16959=ORIENTED_EDGE ( 'NONE', *, *, #152, .T. ) ;
#16960=DIRECTION ( 'NONE',  ( 0.000000000000000000, 1.000000000000000000, 0.000000000000000000 ) ) ;
#16961=DIRECTION ( 'NONE',  ( -4.274815082592931898E-19, -0.9999939076577903929, -0.003490651415223739937 ) ) ;
#16962=DIRECTION ( 'NONE',  ( 0.000000000000000000, 1.000000000000000000, 0.000000000000000000 ) ) ;
#16963=ORIENTED_EDGE ( 'NONE', *, *, #9554, .F. ) ;
#16964=CARTESIAN_POINT ( 'NONE',  ( 3.549999999999944755, 2.500000000000000000, -2.511473670974877948 ) ) ;
#16965=CARTESIAN_POINT ( 'NONE',  ( -14.19999999999998685, 12.50000000000000000, -0.06509327318403752838 ) ) ;
#16968=EDGE_LOOP ( 'NONE', ( #98083, #106977, #79927, #96668 ) ) ;
#16969=AXIS2_PLACEMENT_3D ( 'NONE', #115145, #95547, #56876 ) ;
#16970=CARTESIAN_POINT ( 'NONE',  ( -0.6500000000000389910, 2.500000000000000000, -6.248780366869526759 ) ) ;
#16971=AXIS2_PLACEMENT_3D ( 'NONE', #59682, #17109, #29549 ) ;
#16972=CIRCLE ( 'NONE', #83907, 0.06509327318403745899 ) ;
#16973=LINE ( 'NONE', #67368, #119206 ) ;
#16974=EDGE_CURVE ( 'NONE', #84331, #69984, #81643, .T. ) ;
#16975=AXIS2_PLACEMENT_3D ( 'NONE', #45208, #85115, #106687 ) ;
#16976=AXIS2_PLACEMENT_3D ( 'NONE', #24039, #95995, #63956 ) ;
#16977=CIRCLE ( 'NONE', #23277, 0.06509327318403745899 ) ;
#16978=VERTEX_POINT ( 'NONE', #53602 ) ;
#16979=DIRECTION ( 'NONE',  ( 0.000000000000000000, 0.000000000000000000, 1.000000000000000000 ) ) ;
#16980=DIRECTION ( 'NONE',  ( 0.000000000000000000, 1.000000000000000000, 0.000000000000000000 ) ) ;
#16981=EDGE_CURVE ( 'NONE', #126577, #118519, #33328, .T. ) ;
#16983=FACE_OUTER_BOUND ( 'NONE', #53384, .T. ) ;
#16984=EDGE_CURVE ( 'NONE', #77757, #29713, #41852, .T. ) ;
#16985=ORIENTED_EDGE ( 'NONE', *, *, #1235, .F. ) ;
#16986=LINE ( 'NONE', #77243, #98025 ) ;
#16987=ORIENTED_EDGE ( 'NONE', *, *, #10091, .T. ) ;
#16988=EDGE_CURVE ( 'NONE', #55865, #21250, #27260, .T. ) ;
#16989=EDGE_CURVE ( 'NONE', #82532, #57756, #1267, .T. ) ;
#16990=ORIENTED_EDGE ( 'NONE', *, *, #7587, .F. ) ;
#16991=ORIENTED_EDGE ( 'NONE', *, *, #121472, .F. ) ;
#16992=EDGE_CURVE ( 'NONE', #87403, #21143, #75289, .T. ) ;
#16993=DIRECTION ( 'NONE',  ( 0.000000000000000000, 0.000000000000000000, 1.000000000000000000 ) ) ;
#16994=EDGE_CURVE ( 'NONE', #46254, #121408, #103985, .T. ) ;
#16995=EDGE_CURVE ( 'NONE', #117447, #36746, #85748, .T. ) ;
#16996=FACE_BOUND ( 'NONE', #61400, .T. ) ;
#16997=CARTESIAN_POINT ( 'NONE',  ( -10.20000000000000284, 12.50000000000000000, 4.048810130592458201 ) ) ;
#16998=DIRECTION ( 'NONE',  ( -0.000000000000000000, 1.000000000000000000, -0.000000000000000000 ) ) ;
#16999=DIRECTION ( 'NONE',  ( 0.000000000000000000, 0.000000000000000000, -1.000000000000000000 ) ) ;
#17000=ORIENTED_EDGE ( 'NONE', *, *, #25401, .F. ) ;
#17001=DIRECTION ( 'NONE',  ( -0.000000000000000000, 1.000000000000000000, -0.000000000000000000 ) ) ;
#17002=DIRECTION ( 'NONE',  ( 0.000000000000000000, 0.000000000000000000, -1.000000000000000000 ) ) ;
#17003=EDGE_CURVE ( 'NONE', #108664, #5075, #81127, .T. ) ;
#17004=CARTESIAN_POINT ( 'NONE',  ( -7.100000000000013856, 12.50000000000000000, 3.637306695894644726 ) ) ;
#17005=CARTESIAN_POINT ( 'NONE',  ( -6.450000000000017941, 12.50000000000000000, -2.446380397790840266 ) ) ;
#17006=ORIENTED_EDGE ( 'NONE', *, *, #59383, .F. ) ;
#17007=AXIS2_PLACEMENT_3D ( 'NONE', #84938, #14876, #4414 ) ;
#17008=CARTESIAN_POINT ( 'NONE',  ( -14.14999999999998614, 2.500000000000000000, -2.957883832488651610 ) ) ;
#17009=CARTESIAN_POINT ( 'NONE',  ( -8.550000000000011369, 2.500000000000000000, -2.511473670974877948 ) ) ;
#17010=ORIENTED_EDGE ( 'NONE', *, *, #85978, .T. ) ;
#17011=DIRECTION ( 'NONE',  ( 0.000000000000000000, -0.9999939076577903929, 0.003490651415223739937 ) ) ;
#17012=DIRECTION ( 'NONE',  ( 0.000000000000000000, 0.000000000000000000, -1.000000000000000000 ) ) ;
#17013=FACE_BOUND ( 'NONE', #58329, .T. ) ;
#17014=CIRCLE ( 'NONE', #90202, 0.06509327318403745899 ) ;
#17015=CARTESIAN_POINT ( 'NONE',  ( 7.173569985920785541, -2.500000000000000000, -8.713264184442472526 ) ) ;
#17016=AXIS2_PLACEMENT_3D ( 'NONE', #74615, #107292, #104702 ) ;
#17017=ORIENTED_EDGE ( 'NONE', *, *, #10364, .T. ) ;
#17018=AXIS2_PLACEMENT_3D ( 'NONE', #2333, #20073, #90738 ) ;
#17019=DIRECTION ( 'NONE',  ( 0.000000000000000000, -0.000000000000000000, 1.000000000000000000 ) ) ;
#17020=ORIENTED_EDGE ( 'NONE', *, *, #33062, .F. ) ;
#17021=VERTEX_POINT ( 'NONE', #92211 ) ;
#17022=CARTESIAN_POINT ( 'NONE',  ( 16.86635082839110211, 0.4716143926291168631, -5.778906370536269321 ) ) ;
#17024=ORIENTED_EDGE ( 'NONE', *, *, #25746, .F. ) ;
#17025=AXIS2_PLACEMENT_3D ( 'NONE', #123435, #124084, #25889 ) ;
#17026=CARTESIAN_POINT ( 'NONE',  ( 14.14999999999989200, 2.500000000000000000, -2.265063509461101798 ) ) ;
#17027=DIRECTION ( 'NONE',  ( 0.000000000000000000, -0.000000000000000000, 1.000000000000000000 ) ) ;
#17028=CONICAL_SURFACE ( 'NONE', #98617, 0.1000000000000000472, 0.003490658503988666988 ) ;
#17029=CIRCLE ( 'NONE', #90220, 0.09999999999999999167 ) ;
#17030=CARTESIAN_POINT ( 'NONE',  ( 13.34999999999989662, 12.50000000000000000, -1.472243186433550122 ) ) ;
#17031=EDGE_CURVE ( 'NONE', #43734, #8654, #94167, .T. ) ;
#17033=CONICAL_SURFACE ( 'NONE', #90222, 0.1000000000000002554, 0.003490658503988666988 ) ;
#17034=EDGE_CURVE ( 'NONE', #109486, #16978, #62791, .T. ) ;
#17035=EDGE_LOOP ( 'NONE', ( #5001, #65090, #120774, #126329 ) ) ;
#17036=ADVANCED_FACE ( 'NONE', ( #73233 ), #23076, .T. ) ;
#17037=CARTESIAN_POINT ( 'NONE',  ( 7.899999999999921307, 2.500000000000000000, -0.1000000000000023925 ) ) ;
#17038=CIRCLE ( 'NONE', #10705, 0.1000000000000002554 ) ;
#17039=CIRCLE ( 'NONE', #60994, 0.1000000000000000056 ) ;
#17040=DIRECTION ( 'NONE',  ( 0.000000000000000000, -0.9999939076577903929, 0.003490651415223739937 ) ) ;
#17041=LINE ( 'NONE', #85811, #109813 ) ;
#17042=CARTESIAN_POINT ( 'NONE',  ( -12.69999999999999396, 12.50000000000000000, 0.4115034346978150848 ) ) ;
#17043=ORIENTED_EDGE ( 'NONE', *, *, #67229, .T. ) ;
#17044=PLANE ( 'NONE',  #9856 ) ;
#17045=ORIENTED_EDGE ( 'NONE', *, *, #21019, .F. ) ;
#17046=EDGE_CURVE ( 'NONE', #76513, #79082, #79511, .T. ) ;
#17047=FACE_OUTER_BOUND ( 'NONE', #82379, .T. ) ;
#17048=DIRECTION ( 'NONE',  ( -0.000000000000000000, -1.000000000000000000, -0.000000000000000000 ) ) ;
#17049=ADVANCED_FACE ( 'NONE', ( #23481 ), #151, .T. ) ;
#17050=VERTEX_POINT ( 'NONE', #71956 ) ;
#17051=CARTESIAN_POINT ( 'NONE',  ( -0.4000000000000396572, 12.50000000000000000, 4.330127018922196314 ) ) ;
#17052=DIRECTION ( 'NONE',  ( 0.000000000000000000, 1.000000000000000000, 0.000000000000000000 ) ) ;
#17053=EDGE_CURVE ( 'NONE', #72282, #18843, #54457, .T. ) ;
#17054=DIRECTION ( 'NONE',  ( 0.000000000000000000, 0.000000000000000000, 1.000000000000000000 ) ) ;
#17055=ADVANCED_FACE ( 'NONE', ( #64055 ), #113038, .T. ) ;
#17056=DIRECTION ( 'NONE',  ( -0.000000000000000000, -1.000000000000000000, -0.000000000000000000 ) ) ;
#17057=EDGE_LOOP ( 'NONE', ( #59874, #38521, #112051, #101176 ) ) ;
#17058=FACE_OUTER_BOUND ( 'NONE', #60433, .T. ) ;
#17059=PLANE ( 'NONE',  #123319 ) ;
#17061=DIRECTION ( 'NONE',  ( 0.000000000000000000, 0.000000000000000000, 1.000000000000000000 ) ) ;
#17062=DIRECTION ( 'NONE',  ( -0.000000000000000000, 1.000000000000000000, -0.000000000000000000 ) ) ;
#17063=ADVANCED_FACE ( 'NONE', ( #122345 ), #81728, .T. ) ;
#17064=EDGE_LOOP ( 'NONE', ( #3253, #50345 ) ) ;
#17065=ORIENTED_EDGE ( 'NONE', *, *, #74394, .T. ) ;
#17066=DIRECTION ( 'NONE',  ( 0.000000000000000000, -0.000000000000000000, 1.000000000000000000 ) ) ;
#17067=ORIENTED_EDGE ( 'NONE', *, *, #89792, .F. ) ;
#17068=CONICAL_SURFACE ( 'NONE', #35891, 0.1000000000000002554, 0.003490658503988666988 ) ;
#17069=DIRECTION ( 'NONE',  ( -0.000000000000000000, -1.000000000000000000, -0.000000000000000000 ) ) ;
#17070=CONICAL_SURFACE ( 'NONE', #73527, 0.1000000000000002554, 0.003490658503988666988 ) ;
#17071=CIRCLE ( 'NONE', #117424, 0.06509327318403745899 ) ;
#17072=VERTEX_POINT ( 'NONE', #62778 ) ;
#17073=EDGE_LOOP ( 'NONE', ( #83131, #65394, #5574, #74536 ) ) ;
#17074=ORIENTED_EDGE ( 'NONE', *, *, #102200, .T. ) ;
#17075=DIRECTION ( 'NONE',  ( -0.000000000000000000, -1.000000000000000000, -0.000000000000000000 ) ) ;
#17076=CARTESIAN_POINT ( 'NONE',  ( 10.39999999999991154, 12.50000000000000000, -3.637306695894650055 ) ) ;
#17077=CIRCLE ( 'NONE', #77650, 0.06509327318403745899 ) ;
#17078=FACE_OUTER_BOUND ( 'NONE', #106351, .T. ) ;
#17079=CONICAL_SURFACE ( 'NONE', #27561, 0.09999999999999982514, 0.003490658503988666988 ) ;
#17080=DIRECTION ( 'NONE',  ( 0.000000000000000000, 1.000000000000000000, 0.000000000000000000 ) ) ;
#17081=DIRECTION ( 'NONE',  ( 0.000000000000000000, 0.000000000000000000, 1.000000000000000000 ) ) ;
#17082=AXIS2_PLACEMENT_3D ( 'NONE', #128697, #47529, #117515 ) ;
#17083=CARTESIAN_POINT ( 'NONE',  ( -9.400000000000007461, 12.50000000000000000, -0.3464101615137783474 ) ) ;
#17084=AXIS2_PLACEMENT_3D ( 'NONE', #27629, #96373, #85910 ) ;
#17085=EDGE_CURVE ( 'NONE', #72494, #89288, #108821, .T. ) ;
#17086=ORIENTED_EDGE ( 'NONE', *, *, #86200, .F. ) ;
#17087=DIRECTION ( 'NONE',  ( 0.000000000000000000, 1.000000000000000000, 0.000000000000000000 ) ) ;
#17089=ORIENTED_EDGE ( 'NONE', *, *, #115648, .T. ) ;
#17090=ORIENTED_EDGE ( 'NONE', *, *, #83650, .T. ) ;
#17091=EDGE_LOOP ( 'NONE', ( #106900, #11827, #85613, #84293 ) ) ;
#17092=ORIENTED_EDGE ( 'NONE', *, *, #45553, .T. ) ;
#17093=DIRECTION ( 'NONE',  ( 0.000000000000000000, 0.000000000000000000, 1.000000000000000000 ) ) ;
#17094=VERTEX_POINT ( 'NONE', #96088 ) ;
#17095=VERTEX_POINT ( 'NONE', #54239 ) ;
#17096=DIRECTION ( 'NONE',  ( 0.000000000000000000, 1.000000000000000000, 0.000000000000000000 ) ) ;
#17098=EDGE_CURVE ( 'NONE', #31405, #71950, #94155, .T. ) ;
#17099=DIRECTION ( 'NONE',  ( 0.000000000000000000, -0.000000000000000000, 1.000000000000000000 ) ) ;
#17100=DIRECTION ( 'NONE',  ( 0.000000000000000000, 0.000000000000000000, 1.000000000000000000 ) ) ;
#17101=CARTESIAN_POINT ( 'NONE',  ( -7.900000000000011013, 12.50000000000000000, 3.637306695894644726 ) ) ;
#17102=ORIENTED_EDGE ( 'NONE', *, *, #31428, .F. ) ;
#17103=DIRECTION ( 'NONE',  ( 0.000000000000000000, 0.000000000000000000, 1.000000000000000000 ) ) ;
#17104=AXIS2_PLACEMENT_3D ( 'NONE', #20076, #101852, #404 ) ;
#17105=CIRCLE ( 'NONE', #46372, 0.09999999999999982514 ) ;
#17106=ORIENTED_EDGE ( 'NONE', *, *, #83456, .T. ) ;
#17107=CARTESIAN_POINT ( 'NONE',  ( 2.049999999999950084, 2.500000000000000000, -2.265063509461101798 ) ) ;
#17108=ORIENTED_EDGE ( 'NONE', *, *, #101030, .F. ) ;
#17109=DIRECTION ( 'NONE',  ( -0.000000000000000000, 1.000000000000000000, -0.000000000000000000 ) ) ;
#17110=VERTEX_POINT ( 'NONE', #115721 ) ;
#17111=ADVANCED_FACE ( 'NONE', ( #126195 ), #98356, .T. ) ;
#17112=EDGE_LOOP ( 'NONE', ( #97392, #63245 ) ) ;
#17113=CARTESIAN_POINT ( 'NONE',  ( 7.299999999999926104, 2.500000000000000000, -4.083716857408426826 ) ) ;
#17114=DIRECTION ( 'NONE',  ( 0.000000000000000000, 0.000000000000000000, 1.000000000000000000 ) ) ;
#17115=AXIS2_PLACEMENT_3D ( 'NONE', #95724, #125182, #65608 ) ;
#17117=AXIS2_PLACEMENT_3D ( 'NONE', #93963, #102495, #122151 ) ;
#17118=DIRECTION ( 'NONE',  ( 0.000000000000000000, -0.9999939076577903929, 0.003490651415223739937 ) ) ;
#17119=DIRECTION ( 'NONE',  ( 0.000000000000000000, 0.000000000000000000, -1.000000000000000000 ) ) ;
#17120=ORIENTED_EDGE ( 'NONE', *, *, #113606, .T. ) ;
#17121=CARTESIAN_POINT ( 'NONE',  ( -4.350000000000027178, 2.500000000000000000, -6.048780366869526581 ) ) ;
#17122=CARTESIAN_POINT ( 'NONE',  ( -5.850000000000018296, 12.50000000000000000, 2.857883832488649301 ) ) ;
#17123=DIRECTION ( 'NONE',  ( 0.000000000000000000, 1.000000000000000000, 0.000000000000000000 ) ) ;
#17124=DIRECTION ( 'NONE',  ( 0.000000000000000000, 0.000000000000000000, 1.000000000000000000 ) ) ;
#17125=AXIS2_PLACEMENT_3D ( 'NONE', #43937, #74031, #73373 ) ;
#17126=AXIS2_PLACEMENT_3D ( 'NONE', #50531, #31554, #111377 ) ;
#17127=DIRECTION ( 'NONE',  ( 0.000000000000000000, 0.000000000000000000, 1.000000000000000000 ) ) ;
#17128=EDGE_LOOP ( 'NONE', ( #46452, #128656 ) ) ;
#17129=AXIS2_PLACEMENT_3D ( 'NONE', #118637, #8664, #99661 ) ;
#17130=CONICAL_SURFACE ( 'NONE', #42226, 0.09999999999999982514, 0.003490658503988666988 ) ;
#17131=EDGE_LOOP ( 'NONE', ( #94606, #76102, #78500, #6059 ) ) ;
#17132=CARTESIAN_POINT ( 'NONE',  ( -2.300000000000033573, 12.50000000000000000, 0.4115034346978109769 ) ) ;
#17133=AXIS2_PLACEMENT_3D ( 'NONE', #84015, #96901, #17012 ) ;
#17134=ORIENTED_EDGE ( 'NONE', *, *, #105152, .F. ) ;
#17135=DIRECTION ( 'NONE',  ( 0.000000000000000000, 0.000000000000000000, 1.000000000000000000 ) ) ;
#17136=DIRECTION ( 'NONE',  ( 0.000000000000000000, 0.000000000000000000, -1.000000000000000000 ) ) ;
#17137=EDGE_CURVE ( 'NONE', #30008, #118142, #21093, .T. ) ;
#17138=AXIS2_PLACEMENT_3D ( 'NONE', #7891, #30139, #56983 ) ;
#17139=EDGE_LOOP ( 'NONE', ( #24329, #112993 ) ) ;
#17141=DIRECTION ( 'NONE',  ( -0.000000000000000000, 1.000000000000000000, -0.000000000000000000 ) ) ;
#17142=DIRECTION ( 'NONE',  ( 0.000000000000000000, 0.000000000000000000, -1.000000000000000000 ) ) ;
#17143=DIRECTION ( 'NONE',  ( 0.000000000000000000, 1.000000000000000000, 0.000000000000000000 ) ) ;
#17144=VERTEX_POINT ( 'NONE', #75793 ) ;
#17145=EDGE_CURVE ( 'NONE', #66592, #19145, #73322, .T. ) ;
#17146=CARTESIAN_POINT ( 'NONE',  ( -7.500000000000001776, -1.500000000000000000, 10.00000000000000178 ) ) ;
#17148=ORIENTED_EDGE ( 'NONE', *, *, #129442, .T. ) ;
#17149=EDGE_CURVE ( 'NONE', #72904, #65479, #47004, .T. ) ;
#17150=EDGE_CURVE ( 'NONE', #118811, #91731, #69120, .T. ) ;
#17151=EDGE_CURVE ( 'NONE', #125468, #93533, #126847, .T. ) ;
#17153=ADVANCED_FACE ( 'NONE', ( #124910 ), #104612, .T. ) ;
#17154=CARTESIAN_POINT ( 'NONE',  ( 4.349999999999937472, 2.500000000000000000, 6.841600689897072485 ) ) ;
#17155=DIRECTION ( 'NONE',  ( -4.274815082592931898E-19, -0.9999939076577903929, -0.003490651415223739937 ) ) ;
#17156=ORIENTED_EDGE ( 'NONE', *, *, #47209, .T. ) ;
#17157=DIRECTION ( 'NONE',  ( 0.000000000000000000, 0.000000000000000000, 1.000000000000000000 ) ) ;
#17158=AXIS2_PLACEMENT_3D ( 'NONE', #21398, #90123, #451 ) ;
#17159=AXIS2_PLACEMENT_3D ( 'NONE', #48592, #41366, #9303 ) ;
#17160=CIRCLE ( 'NONE', #29722, 0.1000000000000002554 ) ;
#17162=DIRECTION ( 'NONE',  ( -0.000000000000000000, 1.000000000000000000, -0.000000000000000000 ) ) ;
#17163=CARTESIAN_POINT ( 'NONE',  ( -11.05000000000000071, 2.500000000000000000, -2.511473670974873951 ) ) ;
#17164=EDGE_CURVE ( 'NONE', #45421, #112782, #124270, .T. ) ;
#17165=PLANE ( 'NONE',  #22507 ) ;
#17166=ORIENTED_EDGE ( 'NONE', *, *, #19671, .T. ) ;
#17167=EDGE_CURVE ( 'NONE', #102949, #109829, #55531, .T. ) ;
#17168=AXIS2_PLACEMENT_3D ( 'NONE', #68543, #79033, #91901 ) ;
#17169=FACE_OUTER_BOUND ( 'NONE', #116253, .T. ) ;
#17170=EDGE_CURVE ( 'NONE', #39659, #12221, #115064, .T. ) ;
#17171=VECTOR ( 'NONE', #13765, 1000.000000000000000 ) ;
#17172=CIRCLE ( 'NONE', #40203, 0.1000000000000002554 ) ;
#17173=DIRECTION ( 'NONE',  ( 0.000000000000000000, -0.000000000000000000, 1.000000000000000000 ) ) ;
#17174=CIRCLE ( 'NONE', #36002, 0.06509327318403745899 ) ;
#17175=ORIENTED_EDGE ( 'NONE', *, *, #14501, .F. ) ;
#17176=AXIS2_PLACEMENT_3D ( 'NONE', #127562, #48354, #98095 ) ;
#17177=CARTESIAN_POINT ( 'NONE',  ( 10.84999999999991260, 12.50000000000000000, -2.165063509461101710 ) ) ;
#17178=ORIENTED_EDGE ( 'NONE', *, *, #36383, .T. ) ;
#17179=CIRCLE ( 'NONE', #42270, 0.1000000000000002554 ) ;
#17180=CARTESIAN_POINT ( 'NONE',  ( -13.14999999999999147, 2.500000000000000000, 1.718653347947325383 ) ) ;
#17181=ORIENTED_EDGE ( 'NONE', *, *, #45984, .F. ) ;
#17182=CARTESIAN_POINT ( 'NONE',  ( -11.05000000000000071, 12.50000000000000000, -6.841600689897075149 ) ) ;
#17183=CARTESIAN_POINT ( 'NONE',  ( 14.59999999999989484, 2.500000000000000000, -0.7928203230275542301 ) ) ;
#17184=EDGE_LOOP ( 'NONE', ( #59926, #94832, #69664, #92386 ) ) ;
#17185=EDGE_LOOP ( 'NONE', ( #75782, #46271 ) ) ;
#17186=CARTESIAN_POINT ( 'NONE',  ( -1.250000000000036193, 12.50000000000000000, 5.802370205355744659 ) ) ;
#17187=DIRECTION ( 'NONE',  ( -4.274815082592931898E-19, -0.9999939076577903929, -0.003490651415223739937 ) ) ;
#17188=ORIENTED_EDGE ( 'NONE', *, *, #107016, .F. ) ;
#17189=CARTESIAN_POINT ( 'NONE',  ( -1.900000000000034106, 2.500000000000000000, 0.3464101615137735735 ) ) ;
#17190=CARTESIAN_POINT ( 'NONE',  ( -7.300000000000018474, 2.500000000000000000, -3.883716857408426648 ) ) ;
#17191=DIRECTION ( 'NONE',  ( 0.000000000000000000, 1.000000000000000000, 0.000000000000000000 ) ) ;
#17192=CARTESIAN_POINT ( 'NONE',  ( -11.84999999999999609, 2.500000000000000000, 2.611473670974873151 ) ) ;
#17193=DIRECTION ( 'NONE',  ( 0.000000000000000000, 0.000000000000000000, 1.000000000000000000 ) ) ;
#17194=CARTESIAN_POINT ( 'NONE',  ( 2.099999999999950351, 2.500000000000000000, -5.022947341949754119 ) ) ;
#17195=VECTOR ( 'NONE', #85428, 1000.000000000000000 ) ;
#17196=AXIS2_PLACEMENT_3D ( 'NONE', #128069, #67172, #97952 ) ;
#17197=EDGE_LOOP ( 'NONE', ( #62385, #8576 ) ) ;
#17199=ORIENTED_EDGE ( 'NONE', *, *, #28497, .F. ) ;
#17200=EDGE_LOOP ( 'NONE', ( #42786, #115505 ) ) ;
#17201=FACE_OUTER_BOUND ( 'NONE', #100504, .T. ) ;
#17202=FACE_OUTER_BOUND ( 'NONE', #119976, .T. ) ;
#17203=DIRECTION ( 'NONE',  ( 0.000000000000000000, -0.000000000000000000, 1.000000000000000000 ) ) ;
#17204=EDGE_LOOP ( 'NONE', ( #29989, #109325 ) ) ;
#17205=FACE_BOUND ( 'NONE', #54979, .T. ) ;
#17206=ADVANCED_FACE ( 'NONE', ( #95452 ), #2213, .T. ) ;
#17207=AXIS2_PLACEMENT_3D ( 'NONE', #3043, #111027, #21379 ) ;
#17208=CARTESIAN_POINT ( 'NONE',  ( 10.19999999999991580, 12.50000000000000000, -0.2813168883297409439 ) ) ;
#17209=CARTESIAN_POINT ( 'NONE',  ( 14.54999999999989591, 2.500000000000000000, 2.265063509461097357 ) ) ;
#17211=EDGE_CURVE ( 'NONE', #37472, #35157, #18936, .T. ) ;
#17212=CIRCLE ( 'NONE', #48648, 0.06509327318403745899 ) ;
#17213=CARTESIAN_POINT ( 'NONE',  ( -2.100000000000033840, 12.50000000000000000, 3.702399969078682407 ) ) ;
#17214=AXIS2_PLACEMENT_3D ( 'NONE', #32973, #12013, #72876 ) ;
#17215=DIRECTION ( 'NONE',  ( 0.000000000000000000, 0.000000000000000000, 1.000000000000000000 ) ) ;
#17216=ADVANCED_FACE ( 'NONE', ( #125542 ), #90043, .T. ) ;
#17217=CARTESIAN_POINT ( 'NONE',  ( 0.3999999999999555023, 12.50000000000000000, 4.330127018922196314 ) ) ;
#17218=DIRECTION ( 'NONE',  ( 0.000000000000000000, 1.000000000000000000, 0.000000000000000000 ) ) ;
#17219=CARTESIAN_POINT ( 'NONE',  ( -13.29999999999998828, 12.50000000000000000, 4.265033745738159077 ) ) ;
#17220=CARTESIAN_POINT ( 'NONE',  ( 2.699999999999944666, 12.50000000000000000, 4.676537180435972552 ) ) ;
#17221=CARTESIAN_POINT ( 'NONE',  ( -2.300000000000033573, 12.50000000000000000, -3.983716857408426293 ) ) ;
#17222=CIRCLE ( 'NONE', #50702, 0.06509327318403745899 ) ;
#17223=CARTESIAN_POINT ( 'NONE',  ( 12.49999999999990408, 12.50000000000000000, -3.572213422710612374 ) ) ;
#17224=ADVANCED_FACE ( 'NONE', ( #77100 ), #35688, .T. ) ;
#17225=AXIS2_PLACEMENT_3D ( 'NONE', #9180, #90965, #18984 ) ;
#17226=VERTEX_POINT ( 'NONE', #76456 ) ;
#17227=ORIENTED_EDGE ( 'NONE', *, *, #96378, .F. ) ;
#17228=ORIENTED_EDGE ( 'NONE', *, *, #71233, .F. ) ;
#17229=VECTOR ( 'NONE', #10368, 1000.000000000000000 ) ;
#17230=VERTEX_POINT ( 'NONE', #26710 ) ;
#17231=AXIS2_PLACEMENT_3D ( 'NONE', #80573, #31469, #83778 ) ;
#17232=CIRCLE ( 'NONE', #115530, 0.09999999999999982514 ) ;
#17233=CARTESIAN_POINT ( 'NONE',  ( 17.50000000000000355, -2.413244906436780024, -3.595454705092401504 ) ) ;
#17234=DIRECTION ( 'NONE',  ( 0.000000000000000000, 1.000000000000000000, 0.000000000000000000 ) ) ;
#17235=VERTEX_POINT ( 'NONE', #66620 ) ;
#17236=ORIENTED_EDGE ( 'NONE', *, *, #9480, .T. ) ;
#17237=ORIENTED_EDGE ( 'NONE', *, *, #1867, .F. ) ;
#17238=AXIS2_PLACEMENT_3D ( 'NONE', #37204, #77119, #67254 ) ;
#17239=DIRECTION ( 'NONE',  ( -0.000000000000000000, -1.000000000000000000, -0.000000000000000000 ) ) ;
#17240=AXIS2_PLACEMENT_3D ( 'NONE', #64728, #66021, #75201 ) ;
#17241=CARTESIAN_POINT ( 'NONE',  ( -9.800000000000004263, 2.500000000000000000, 3.983716857408420076 ) ) ;
#17242=DIRECTION ( 'NONE',  ( -4.274815082592931898E-19, -0.9999939076577903929, -0.003490651415223739937 ) ) ;
#17243=LINE ( 'NONE', #125924, #88963 ) ;
#17244=PLANE ( 'NONE',  #39386 ) ;
#17245=ADVANCED_FACE ( 'NONE', ( #16847 ), #116997, .T. ) ;
#17246=ORIENTED_EDGE ( 'NONE', *, *, #94708, .F. ) ;
#17247=EDGE_LOOP ( 'NONE', ( #42993, #99985, #56194, #59557 ) ) ;
#17248=ORIENTED_EDGE ( 'NONE', *, *, #75410, .F. ) ;
#17249=VERTEX_POINT ( 'NONE', #27995 ) ;
#17250=CARTESIAN_POINT ( 'NONE',  ( -12.89999999999999147, 2.500000000000000000, -0.5928203230275499447 ) ) ;
#17251=CONICAL_SURFACE ( 'NONE', #59056, 0.1000000000000002554, 0.003490658503988666988 ) ;
#17252=VERTEX_POINT ( 'NONE', #47642 ) ;
#17253=EDGE_LOOP ( 'NONE', ( #82987, #127167, #39361, #108474 ) ) ;
#17254=CARTESIAN_POINT ( 'NONE',  ( -8.550000000000013145, 2.500000000000000000, -1.818653347947326138 ) ) ;
#17255=CARTESIAN_POINT ( 'NONE',  ( 3.099999999999945466, 12.50000000000000000, 0.3464101615137735735 ) ) ;
#17256=CARTESIAN_POINT ( 'NONE',  ( -6.450000000000017941, 2.500000000000000000, -2.511473670974877948 ) ) ;
#17257=ADVANCED_FACE ( 'NONE', ( #67914 ), #87977, .T. ) ;
#17258=CIRCLE ( 'NONE', #46520, 0.1000000000000002554 ) ;
#17259=DIRECTION ( 'NONE',  ( -0.000000000000000000, 1.000000000000000000, -0.000000000000000000 ) ) ;
#17260=AXIS2_PLACEMENT_3D ( 'NONE', #85678, #77157, #84394 ) ;
#17261=VECTOR ( 'NONE', #5858, 1000.000000000000000 ) ;
#17262=CARTESIAN_POINT ( 'NONE',  ( -9.600000000000006750, 2.500000000000000000, 3.637306695894644726 ) ) ;
#17263=ORIENTED_EDGE ( 'NONE', *, *, #501, .F. ) ;
#17264=DIRECTION ( 'NONE',  ( 0.000000000000000000, 0.000000000000000000, -1.000000000000000000 ) ) ;
#17265=CIRCLE ( 'NONE', #31879, 0.1000000000000000056 ) ;
#17266=AXIS2_PLACEMENT_3D ( 'NONE', #105876, #126809, #75757 ) ;
#17267=VERTEX_POINT ( 'NONE', #69190 ) ;
#17268=DIRECTION ( 'NONE',  ( 0.000000000000000000, 0.000000000000000000, -1.000000000000000000 ) ) ;
#17269=VECTOR ( 'NONE', #64486, 1000.000000000000000 ) ;
#17270=EDGE_LOOP ( 'NONE', ( #123824, #100918 ) ) ;
#17272=DIRECTION ( 'NONE',  ( 0.000000000000000000, -0.9999939076577903929, 0.003490651415223739937 ) ) ;
#17273=VERTEX_POINT ( 'NONE', #98016 ) ;
#17274=CIRCLE ( 'NONE', #90440, 0.09999999999999982514 ) ;
#17275=CARTESIAN_POINT ( 'NONE',  ( -9.800000000000006040, 12.50000000000000000, 4.611443907251934426 ) ) ;
#17276=AXIS2_PLACEMENT_3D ( 'NONE', #2440, #42395, #122248 ) ;
#17277=EDGE_CURVE ( 'NONE', #83264, #118052, #62876, .T. ) ;
#17279=ORIENTED_EDGE ( 'NONE', *, *, #122695, .F. ) ;
#17280=CIRCLE ( 'NONE', #71689, 0.06509327318403741736 ) ;
#17281=DIRECTION ( 'NONE',  ( 0.000000000000000000, 0.000000000000000000, 1.000000000000000000 ) ) ;
#17282=EDGE_LOOP ( 'NONE', ( #85462, #127230, #105432, #77362 ) ) ;
#17283=ADVANCED_FACE ( 'NONE', ( #48283 ), #8985, .T. ) ;
#17284=EDGE_LOOP ( 'NONE', ( #115854, #563 ) ) ;
#17285=CARTESIAN_POINT ( 'NONE',  ( 4.549999999999939426, 12.50000000000000000, -2.165063509461101710 ) ) ;
#17286=DIRECTION ( 'NONE',  ( 0.000000000000000000, 0.000000000000000000, -1.000000000000000000 ) ) ;
#17288=CARTESIAN_POINT ( 'NONE',  ( 13.34999999999989662, 2.500000000000000000, -2.165063509461101710 ) ) ;
#17290=CARTESIAN_POINT ( 'NONE',  ( -1.250000000000035749, 2.500000000000000000, -2.757883832488654097 ) ) ;
#17291=AXIS2_PLACEMENT_3D ( 'NONE', #53887, #3498, #93816 ) ;
#17292=VERTEX_POINT ( 'NONE', #90115 ) ;
#17293=CONICAL_SURFACE ( 'NONE', #46872, 0.1000000000000002554, 0.003490658503988666988 ) ;
#17294=CARTESIAN_POINT ( 'NONE',  ( -3.150000000000030109, 2.500000000000000000, 1.818653347947321475 ) ) ;
#17295=FACE_OUTER_BOUND ( 'NONE', #124701, .T. ) ;
#17297=EDGE_CURVE ( 'NONE', #83209, #67824, #4346, .T. ) ;
#17298=EDGE_LOOP ( 'NONE', ( #26971, #12330, #99023, #18050 ) ) ;
#17299=DIRECTION ( 'NONE',  ( 0.000000000000000000, -0.000000000000000000, 1.000000000000000000 ) ) ;
#17300=LINE ( 'NONE', #108918, #78219 ) ;
#17301=FACE_OUTER_BOUND ( 'NONE', #53614, .T. ) ;
#17302=CARTESIAN_POINT ( 'NONE',  ( 0.7999999999999548583, 12.50000000000000000, 4.330127018922196314 ) ) ;
#17303=CIRCLE ( 'NONE', #59217, 0.1000000000000002554 ) ;
#17304=CARTESIAN_POINT ( 'NONE',  ( 3.549999999999943867, 12.50000000000000000, -1.753560074763288679 ) ) ;
#17305=AXIS2_PLACEMENT_3D ( 'NONE', #73468, #113401, #63673 ) ;
#17306=ORIENTED_EDGE ( 'NONE', *, *, #117101, .F. ) ;
#17308=EDGE_CURVE ( 'NONE', #64742, #129259, #80328, .T. ) ;
#17309=AXIS2_PLACEMENT_3D ( 'NONE', #36186, #106206, #57093 ) ;
#17310=DIRECTION ( 'NONE',  ( 0.000000000000000000, 0.000000000000000000, 1.000000000000000000 ) ) ;
#17312=ADVANCED_FACE ( 'NONE', ( #444 ), #67044, .T. ) ;
#17313=EDGE_CURVE ( 'NONE', #38667, #108868, #29428, .T. ) ;
#17314=EDGE_CURVE ( 'NONE', #104775, #51072, #40413, .T. ) ;
#17315=ADVANCED_FACE ( 'NONE', ( #88173 ), #104710, .T. ) ;
#17316=AXIS2_PLACEMENT_3D ( 'NONE', #124273, #56155, #27331 ) ;
#17317=EDGE_LOOP ( 'NONE', ( #10455, #113612, #86877, #9161 ) ) ;
#17318=DIRECTION ( 'NONE',  ( -0.000000000000000000, -1.000000000000000000, -0.000000000000000000 ) ) ;
#17319=CIRCLE ( 'NONE', #50506, 0.06509327318403745899 ) ;
#17320=ORIENTED_EDGE ( 'NONE', *, *, #32738, .F. ) ;
#17321=CIRCLE ( 'NONE', #123948, 0.1000000000000000056 ) ;
#17322=VECTOR ( 'NONE', #73007, 1000.000000000000000 ) ;
#17323=VERTEX_POINT ( 'NONE', #109782 ) ;
#17324=CARTESIAN_POINT ( 'NONE',  ( -2.100000000000033396, 2.500000000000000000, -4.922947341949753586 ) ) ;
#17325=ADVANCED_FACE ( 'NONE', ( #39139 ), #37827, .T. ) ;
#17326=ADVANCED_FACE ( 'NONE', ( #20111 ), #48295, .T. ) ;
#17327=AXIS2_PLACEMENT_3D ( 'NONE', #62001, #101915, #12229 ) ;
#17328=ORIENTED_EDGE ( 'NONE', *, *, #18385, .F. ) ;
#17329=DIRECTION ( 'NONE',  ( 0.000000000000000000, -0.9999939076577903929, 0.003490651415223739937 ) ) ;
#17330=CARTESIAN_POINT ( 'NONE',  ( -13.94999999999998685, 2.500000000000000000, 1.718653347947325383 ) ) ;
#17331=DIRECTION ( 'NONE',  ( 0.000000000000000000, 0.000000000000000000, -1.000000000000000000 ) ) ;
#17332=ORIENTED_EDGE ( 'NONE', *, *, #16176, .T. ) ;
#17333=ADVANCED_FACE ( 'NONE', ( #79670 ), #7696, .T. ) ;
#17334=FACE_BOUND ( 'NONE', #79686, .T. ) ;
#17335=ADVANCED_FACE ( 'NONE', ( #79047 ), #117297, .T. ) ;
#17336=AXIS2_PLACEMENT_3D ( 'NONE', #17554, #66652, #79084 ) ;
#17337=CARTESIAN_POINT ( 'NONE',  ( 3.349999999999944578, 2.500000000000000000, -5.802370205355749988 ) ) ;
#17338=ORIENTED_EDGE ( 'NONE', *, *, #95880, .F. ) ;
#17340=EDGE_CURVE ( 'NONE', #94540, #46019, #67131, .T. ) ;
#17341=CARTESIAN_POINT ( 'NONE',  ( -15.59999999999998010, 2.500000000000000000, 0.4464101615137759382 ) ) ;
#17342=ADVANCED_FACE ( 'NONE', ( #49587 ), #12765, .T. ) ;
#17343=ORIENTED_EDGE ( 'NONE', *, *, #23538, .T. ) ;
#17344=ORIENTED_EDGE ( 'NONE', *, *, #99561, .T. ) ;
#17346=LINE ( 'NONE', #116847, #46309 ) ;
#17347=CARTESIAN_POINT ( 'NONE',  ( 3.349999999999941913, 2.500000000000000000, 5.802370205355744659 ) ) ;
#17348=CIRCLE ( 'NONE', #123975, 0.09999999999999982514 ) ;
#17349=CARTESIAN_POINT ( 'NONE',  ( 13.09999999999990195, 2.500000000000000000, 4.576537180435972019 ) ) ;
#17350=CIRCLE ( 'NONE', #94632, 0.09999999999999982514 ) ;
#17351=FACE_BOUND ( 'NONE', #93381, .T. ) ;
#17352=VERTEX_POINT ( 'NONE', #20752 ) ;
#17353=PLANE ( 'NONE',  #117973 ) ;
#17354=FACE_OUTER_BOUND ( 'NONE', #75541, .T. ) ;
#17355=ORIENTED_EDGE ( 'NONE', *, *, #57587, .F. ) ;
#17356=AXIS2_PLACEMENT_3D ( 'NONE', #27170, #7521, #68378 ) ;
#17357=FACE_OUTER_BOUND ( 'NONE', #32864, .T. ) ;
#17358=AXIS2_PLACEMENT_3D ( 'NONE', #88363, #127663, #124611 ) ;
#17359=AXIS2_PLACEMENT_3D ( 'NONE', #8399, #129509, #49003 ) ;
#17360=DIRECTION ( 'NONE',  ( 0.000000000000000000, 0.000000000000000000, 1.000000000000000000 ) ) ;
#17361=AXIS2_PLACEMENT_3D ( 'NONE', #31175, #52724, #63194 ) ;
#17362=DIRECTION ( 'NONE',  ( -0.000000000000000000, -1.000000000000000000, -0.000000000000000000 ) ) ;
#17363=CARTESIAN_POINT ( 'NONE',  ( -9.400000000000007461, 12.50000000000000000, 0.3464101615137735735 ) ) ;
#17364=DIRECTION ( 'NONE',  ( 0.000000000000000000, 0.000000000000000000, 1.000000000000000000 ) ) ;
#17365=AXIS2_PLACEMENT_3D ( 'NONE', #58405, #98297, #8616 ) ;
#17366=AXIS2_PLACEMENT_3D ( 'NONE', #44371, #104581, #35221 ) ;
#17367=AXIS2_PLACEMENT_3D ( 'NONE', #32970, #12010, #32332 ) ;
#17368=ORIENTED_EDGE ( 'NONE', *, *, #45686, .F. ) ;
#17369=ORIENTED_EDGE ( 'NONE', *, *, #118129, .F. ) ;
#17370=ORIENTED_EDGE ( 'NONE', *, *, #53680, .T. ) ;
#17371=ORIENTED_EDGE ( 'NONE', *, *, #125056, .F. ) ;
#17372=AXIS2_PLACEMENT_3D ( 'NONE', #7760, #512, #40477 ) ;
#17373=ORIENTED_EDGE ( 'NONE', *, *, #102734, .T. ) ;
#17374=LINE ( 'NONE', #19315, #58898 ) ;
#17375=CARTESIAN_POINT ( 'NONE',  ( -4.600000000000028066, 12.50000000000000000, -3.637306695894650055 ) ) ;
#17376=ORIENTED_EDGE ( 'NONE', *, *, #99772, .T. ) ;
#17377=FACE_BOUND ( 'NONE', #6657, .T. ) ;
#17378=DIRECTION ( 'NONE',  ( 0.000000000000000000, 0.000000000000000000, -1.000000000000000000 ) ) ;
#17379=ADVANCED_FACE ( 'NONE', ( #60693 ), #2301, .T. ) ;
#17380=FACE_OUTER_BOUND ( 'NONE', #16140, .T. ) ;
#17381=ADVANCED_FACE ( 'NONE', ( #71133 ), #80968, .T. ) ;
#17382=CARTESIAN_POINT ( 'NONE',  ( -1.250000000000001110, 2.500000000000000000, -2.165063509461101710 ) ) ;
#17383=CARTESIAN_POINT ( 'NONE',  ( -1.850000000000033396, 12.50000000000000000, -1.818653347947325916 ) ) ;
#17384=FACE_OUTER_BOUND ( 'NONE', #80984, .T. ) ;
#17385=VERTEX_POINT ( 'NONE', #122185 ) ;
#17386=CARTESIAN_POINT ( 'NONE',  ( 18.00406198521865164, -1.510509990005264314, 4.944015973543655740 ) ) ;
#17387=CIRCLE ( 'NONE', #13183, 0.06509327318403745899 ) ;
#17388=ADVANCED_FACE ( 'NONE', ( #83550 ), #115160, .T. ) ;
#17389=VERTEX_POINT ( 'NONE', #22704 ) ;
#17390=ORIENTED_EDGE ( 'NONE', *, *, #70778, .F. ) ;
#17391=ORIENTED_EDGE ( 'NONE', *, *, #62884, .F. ) ;
#17392=DIRECTION ( 'NONE',  ( 0.000000000000000000, 0.000000000000000000, 1.000000000000000000 ) ) ;
#17394=CARTESIAN_POINT ( 'NONE',  ( -7.500000000000001776, -1.500000000000000000, 9.000000000000001776 ) ) ;
#17395=ORIENTED_EDGE ( 'NONE', *, *, #32195, .F. ) ;
#17396=CARTESIAN_POINT ( 'NONE',  ( 4.912722231850285226, 2.500000000000252687, -9.942384338124218957 ) ) ;
#17397=AXIS2_PLACEMENT_3D ( 'NONE', #97993, #27308, #56132 ) ;
#17399=CONICAL_SURFACE ( 'NONE', #52933, 0.1000000000000002554, 0.003490658503988666988 ) ;
#17400=CARTESIAN_POINT ( 'NONE',  ( 3.149999999999942624, 2.500000000000000000, 6.148780366869520897 ) ) ;
#17401=CARTESIAN_POINT ( 'NONE',  ( -12.29999999999999361, 12.50000000000000000, 3.983716857408420076 ) ) ;
#17403=DIRECTION ( 'NONE',  ( 0.000000000000000000, 0.000000000000000000, -1.000000000000000000 ) ) ;
#17404=FACE_OUTER_BOUND ( 'NONE', #7710, .T. ) ;
#17405=DIRECTION ( 'NONE',  ( 0.000000000000000000, -0.9999939076577903929, 0.003490651415223739937 ) ) ;
#17406=VECTOR ( 'NONE', #128965, 1000.000000000000000 ) ;
#17407=ORIENTED_EDGE ( 'NONE', *, *, #10221, .T. ) ;
#17408=DIRECTION ( 'NONE',  ( -0.000000000000000000, -1.000000000000000000, -0.000000000000000000 ) ) ;
#17409=CIRCLE ( 'NONE', #98902, 0.06509327318403745899 ) ;
#17410=CIRCLE ( 'NONE', #63406, 0.06509327318403745899 ) ;
#17411=ORIENTED_EDGE ( 'NONE', *, *, #56473, .F. ) ;
#17412=VECTOR ( 'NONE', #51804, 1000.000000000000000 ) ;
#17413=ORIENTED_EDGE ( 'NONE', *, *, #84151, .T. ) ;
#17414=CARTESIAN_POINT ( 'NONE',  ( -3.950000000000024603, 12.50000000000000000, -2.511473670974877948 ) ) ;
#17415=FACE_OUTER_BOUND ( 'NONE', #101762, .T. ) ;
#17416=DIRECTION ( 'NONE',  ( 0.000000000000000000, 0.000000000000000000, 1.000000000000000000 ) ) ;
#17417=AXIS2_PLACEMENT_3D ( 'NONE', #67440, #87743, #59618 ) ;
#17418=ORIENTED_EDGE ( 'NONE', *, *, #53674, .T. ) ;
#17419=VERTEX_POINT ( 'NONE', #61973 ) ;
#17420=EDGE_CURVE ( 'NONE', #3252, #30644, #90126, .T. ) ;
#17421=CARTESIAN_POINT ( 'NONE',  ( 10.44999999999991402, 2.500000000000000000, -2.165063509461101710 ) ) ;
#17422=CARTESIAN_POINT ( 'NONE',  ( -12.04999999999999716, 2.500000000000000000, -6.395190528383298378 ) ) ;
#17423=AXIS2_PLACEMENT_3D ( 'NONE', #29158, #108334, #69055 ) ;
#17424=VECTOR ( 'NONE', #104523, 1000.000000000000000 ) ;
#17425=CARTESIAN_POINT ( 'NONE',  ( -13.54999999999998828, 12.50000000000000000, -2.511473670974875727 ) ) ;
#17426=ORIENTED_EDGE ( 'NONE', *, *, #108506, .T. ) ;
#17427=VERTEX_POINT ( 'NONE', #102528 ) ;
#17428=CARTESIAN_POINT ( 'NONE',  ( 1.249999999999986899, 2.500000000000000000, 6.495190528383297135 ) ) ;
#17429=CIRCLE ( 'NONE', #27916, 0.09999999999999982514 ) ;
#17431=DIRECTION ( 'NONE',  ( -0.000000000000000000, -1.000000000000000000, -0.000000000000000000 ) ) ;
#17432=DIRECTION ( 'NONE',  ( 0.000000000000000000, 1.000000000000000000, 0.000000000000000000 ) ) ;
#17433=ORIENTED_EDGE ( 'NONE', *, *, #5934, .F. ) ;
#17434=CARTESIAN_POINT ( 'NONE',  ( 14.34999999999989662, 2.500000000000000000, 1.818653347947321475 ) ) ;
#17435=DIRECTION ( 'NONE',  ( 0.000000000000000000, 1.000000000000000000, 0.000000000000000000 ) ) ;
#17436=CARTESIAN_POINT ( 'NONE',  ( -2.700000000000031264, 2.500000000000000000, 4.576537180435972019 ) ) ;
#17437=B_SPLINE_CURVE_WITH_KNOTS ( 'NONE', 3,
 ( #128445, #129095, #21039, #100257, #100879, #59708, #70153, #11211, #29569, #99615, #104, #49879, #9933, #41350, #88481, #60959 ),
 .UNSPECIFIED., .F., .F.,
 ( 4, 2, 2, 2, 2, 2, 2, 4 ),
 ( 0.0007527720032625739898, 0.001260609959358783812, 0.001768447915454993743, 0.002022366893503097299, 0.002276285871551201288, 0.002784123827647406665, 0.003799799739839814817, 0.004815475652032223837 ),
 .UNSPECIFIED. ) ;
#17438=EDGE_CURVE ( 'NONE', #116494, #39604, #77616, .T. ) ;
#17439=ADVANCED_FACE ( 'NONE', ( #100588 ), #101894, .T. ) ;
#17440=CARTESIAN_POINT ( 'NONE',  ( -0.6500000000000403233, 2.500000000000000000, 6.148780366869520009 ) ) ;
#17441=EDGE_LOOP ( 'NONE', ( #58935, #110328, #67057, #4975 ) ) ;
#17442=CARTESIAN_POINT ( 'NONE',  ( -0.6500000000000398792, 2.500000000000000000, -2.611473670974877592 ) ) ;
#17443=FACE_OUTER_BOUND ( 'NONE', #96854, .T. ) ;
#17444=VERTEX_POINT ( 'NONE', #43633 ) ;
#17445=VERTEX_POINT ( 'NONE', #3055 ) ;
#17446=AXIS2_PLACEMENT_3D ( 'NONE', #47730, #85702, #116446 ) ;
#17447=AXIS2_PLACEMENT_3D ( 'NONE', #109238, #30720, #119078 ) ;
#17448=EDGE_CURVE ( 'NONE', #36869, #113352, #29519, .T. ) ;
#17449=DIRECTION ( 'NONE',  ( -0.000000000000000000, 1.000000000000000000, -0.000000000000000000 ) ) ;
#17450=DIRECTION ( 'NONE',  ( 0.000000000000000000, 0.000000000000000000, 1.000000000000000000 ) ) ;
#17451=CARTESIAN_POINT ( 'NONE',  ( 1.249999999999988898, 2.500000000000000000, -6.395190528383301931 ) ) ;
#17452=DIRECTION ( 'NONE',  ( 0.000000000000000000, 0.000000000000000000, 1.000000000000000000 ) ) ;
#17453=CARTESIAN_POINT ( 'NONE',  ( -3.350000000000031619, 12.50000000000000000, -5.737276932171712751 ) ) ;
#17454=DIRECTION ( 'NONE',  ( 0.000000000000000000, 0.000000000000000000, 1.000000000000000000 ) ) ;
#17455=CONICAL_SURFACE ( 'NONE', #4842, 0.1000000000000000472, 0.003490658503988666988 ) ;
#17456=AXIS2_PLACEMENT_3D ( 'NONE', #24084, #14865, #92831 ) ;
#17457=DIRECTION ( 'NONE',  ( 0.000000000000000000, -0.9999939076577903929, 0.003490651415223739937 ) ) ;
#17458=VECTOR ( 'NONE', #54264, 1000.000000000000000 ) ;
#17459=CARTESIAN_POINT ( 'NONE',  ( 13.14999999999989733, 12.50000000000000000, -1.883746621131363375 ) ) ;
#17460=DIRECTION ( 'NONE',  ( 0.000000000000000000, 0.000000000000000000, 1.000000000000000000 ) ) ;
#17461=CONICAL_SURFACE ( 'NONE', #94839, 0.09999999999999982514, 0.003490658503988666988 ) ;
#17462=AXIS2_PLACEMENT_3D ( 'NONE', #125806, #33591, #76085 ) ;
#17463=DIRECTION ( 'NONE',  ( -0.000000000000000000, -1.000000000000000000, -0.000000000000000000 ) ) ;
#17464=VECTOR ( 'NONE', #73450, 1000.000000000000000 ) ;
#17465=CIRCLE ( 'NONE', #113630, 0.06509327318403745899 ) ;
#17466=ORIENTED_EDGE ( 'NONE', *, *, #79554, .F. ) ;
#17467=CARTESIAN_POINT ( 'NONE',  ( 8.349999999999923261, 2.500000000000000000, 2.857883832488649301 ) ) ;
#17468=CIRCLE ( 'NONE', #92816, 0.06509327318403745899 ) ;
#17469=DIRECTION ( 'NONE',  ( 0.000000000000000000, 1.000000000000000000, 0.000000000000000000 ) ) ;
#17470=DIRECTION ( 'NONE',  ( 0.000000000000000000, 0.000000000000000000, 1.000000000000000000 ) ) ;
#17471=DIRECTION ( 'NONE',  ( 0.000000000000000000, 0.000000000000000000, -1.000000000000000000 ) ) ;
#17473=DIRECTION ( 'NONE',  ( 0.000000000000000000, -0.000000000000000000, 1.000000000000000000 ) ) ;
#17474=EDGE_CURVE ( 'NONE', #65281, #19309, #98535, .T. ) ;
#17476=CARTESIAN_POINT ( 'NONE',  ( 13.54999999999989768, 2.500000000000000000, -2.511473670974877948 ) ) ;
#17477=ORIENTED_EDGE ( 'NONE', *, *, #161, .F. ) ;
#17478=EDGE_CURVE ( 'NONE', #114104, #25583, #52483, .T. ) ;
#17479=EDGE_CURVE ( 'NONE', #85979, #38146, #50862, .T. ) ;
#17480=CIRCLE ( 'NONE', #109443, 0.06509327318403745899 ) ;
#17481=ORIENTED_EDGE ( 'NONE', *, *, #9103, .F. ) ;
#17482=EDGE_LOOP ( 'NONE', ( #110612, #51771 ) ) ;
#17483=VERTEX_POINT ( 'NONE', #31866 ) ;
#17484=ORIENTED_EDGE ( 'NONE', *, *, #47074, .T. ) ;
#17485=DIRECTION ( 'NONE',  ( -4.274815082592931898E-19, -0.9999939076577903929, -0.003490651415223739937 ) ) ;
#17486=EDGE_CURVE ( 'NONE', #112609, #24484, #121526, .T. ) ;
#17487=ADVANCED_FACE ( 'NONE', ( #52149 ), #1105, .T. ) ;
#17488=ADVANCED_FACE ( 'NONE', ( #82904 ), #37919, .T. ) ;
#17489=AXIS2_PLACEMENT_3D ( 'NONE', #129429, #70474, #120861 ) ;
#17490=FACE_OUTER_BOUND ( 'NONE', #2674, .T. ) ;
#17491=PLANE ( 'NONE',  #31656 ) ;
#17492=CIRCLE ( 'NONE', #111603, 0.06509327318403745899 ) ;
#17493=CARTESIAN_POINT ( 'NONE',  ( -12.09999999999999609, 2.500000000000000000, -4.330127018922198978 ) ) ;
#17494=CIRCLE ( 'NONE', #30049, 0.1000000000000002554 ) ;
#17495=ORIENTED_EDGE ( 'NONE', *, *, #91527, .T. ) ;
#17496=EDGE_CURVE ( 'NONE', #13248, #9486, #91425, .T. ) ;
#17497=CARTESIAN_POINT ( 'NONE',  ( 9.549999999999918998, 2.500000000000000000, 2.265063509461097357 ) ) ;
#17498=ORIENTED_EDGE ( 'NONE', *, *, #37404, .F. ) ;
#17499=CARTESIAN_POINT ( 'NONE',  ( 81.97643238337541050, -3.858501996648050714, -6.173828409589621202 ) ) ;
#17500=CARTESIAN_POINT ( 'NONE',  ( 12.64862127267602254, -2.500000000000000000, -8.430718249867293679 ) ) ;
#17501=DIRECTION ( 'NONE',  ( -0.000000000000000000, -1.000000000000000000, -0.000000000000000000 ) ) ;
#17502=DIRECTION ( 'NONE',  ( 0.000000000000000000, 0.000000000000000000, 1.000000000000000000 ) ) ;
#17503=DIRECTION ( 'NONE',  ( 0.000000000000000000, 0.000000000000000000, -1.000000000000000000 ) ) ;
#17504=CIRCLE ( 'NONE', #90678, 0.1000000000000002554 ) ;
#17505=AXIS2_PLACEMENT_3D ( 'NONE', #88106, #79609, #28577 ) ;
#17506=ADVANCED_FACE ( 'NONE', ( #23313 ), #71793, .T. ) ;
#17507=CONICAL_SURFACE ( 'NONE', #119930, 0.1000000000000002554, 0.003490658503988666988 ) ;
#17508=ORIENTED_EDGE ( 'NONE', *, *, #38366, .F. ) ;
#17510=ORIENTED_EDGE ( 'NONE', *, *, #52986, .F. ) ;
#17511=VERTEX_POINT ( 'NONE', #46848 ) ;
#17512=VERTEX_POINT ( 'NONE', #75012 ) ;
#17513=DIRECTION ( 'NONE',  ( -4.274815082592931898E-19, -0.9999939076577903929, -0.003490651415223739937 ) ) ;
#17514=DIRECTION ( 'NONE',  ( -0.000000000000000000, 1.000000000000000000, -0.000000000000000000 ) ) ;
#17515=CARTESIAN_POINT ( 'NONE',  ( 0.6499999999999566125, 2.500000000000000000, -6.148780366869526226 ) ) ;
#17516=FACE_BOUND ( 'NONE', #107881, .T. ) ;
#17517=CIRCLE ( 'NONE', #42598, 0.06509327318403745899 ) ;
#17518=DIRECTION ( 'NONE',  ( 0.000000000000000000, 1.000000000000000000, 0.000000000000000000 ) ) ;
#17519=CARTESIAN_POINT ( 'NONE',  ( 5.399999999999932854, 12.50000000000000000, 5.088040615133786027 ) ) ;
#17520=DIRECTION ( 'NONE',  ( 0.000000000000000000, 0.000000000000000000, -1.000000000000000000 ) ) ;
#17521=FACE_OUTER_BOUND ( 'NONE', #25525, .T. ) ;
#17522=CIRCLE ( 'NONE', #15463, 0.1000000000000002554 ) ;
#17523=VECTOR ( 'NONE', #68751, 1000.000000000000000 ) ;
#17524=AXIS2_PLACEMENT_3D ( 'NONE', #18725, #97927, #28555 ) ;
#17527=CIRCLE ( 'NONE', #38497, 0.09999999999999982514 ) ;
#17528=CARTESIAN_POINT ( 'NONE',  ( -4.600000000000025402, 2.500000000000000000, -2.385244779468109755E-15 ) ) ;
#17529=AXIS2_PLACEMENT_3D ( 'NONE', #103683, #25749, #4159 ) ;
#17530=CARTESIAN_POINT ( 'NONE',  ( 11.44999999999990692, 2.500000000000000000, -6.841600689897078702 ) ) ;
#17531=ORIENTED_EDGE ( 'NONE', *, *, #38142, .F. ) ;
#17532=ORIENTED_EDGE ( 'NONE', *, *, #49299, .T. ) ;
#17534=ORIENTED_EDGE ( 'NONE', *, *, #110600, .F. ) ;
#17536=FACE_BOUND ( 'NONE', #73248, .T. ) ;
#17537=DIRECTION ( 'NONE',  ( 0.000000000000000000, -0.000000000000000000, 1.000000000000000000 ) ) ;
#17538=DIRECTION ( 'NONE',  ( -0.000000000000000000, 1.000000000000000000, -0.000000000000000000 ) ) ;
#17539=EDGE_CURVE ( 'NONE', #94776, #61381, #73411, .T. ) ;
#17540=AXIS2_PLACEMENT_3D ( 'NONE', #50958, #12925, #63984 ) ;
#17541=ORIENTED_EDGE ( 'NONE', *, *, #22244, .T. ) ;
#17542=CARTESIAN_POINT ( 'NONE',  ( -6.650000000000014566, 2.500000000000000000, 6.595190528383296780 ) ) ;
#17543=VECTOR ( 'NONE', #123639, 1000.000000000000000 ) ;
#17544=CARTESIAN_POINT ( 'NONE',  ( 1.649999999999951950, 2.500000000000000000, -5.802370205355749988 ) ) ;
#17545=PLANE ( 'NONE',  #26483 ) ;
#17546=VERTEX_POINT ( 'NONE', #94001 ) ;
#17548=DIRECTION ( 'NONE',  ( 0.000000000000000000, 0.000000000000000000, 1.000000000000000000 ) ) ;
#17549=EDGE_CURVE ( 'NONE', #63883, #21550, #33712, .T. ) ;
#17550=AXIS2_PLACEMENT_3D ( 'NONE', #63075, #42828, #52605 ) ;
#17551=CONICAL_SURFACE ( 'NONE', #74005, 0.09999999999999999167, 0.003490658503988666988 ) ;
#17552=VECTOR ( 'NONE', #21969, 1000.000000000000000 ) ;
#17553=VERTEX_POINT ( 'NONE', #44245 ) ;
#17554=CARTESIAN_POINT ( 'NONE',  ( 8.099999999999921485, 12.50000000000000000, -0.3464101615137783474 ) ) ;
#17555=CARTESIAN_POINT ( 'NONE',  ( 2.099999999999947686, 12.50000000000000000, 5.022947341949748790 ) ) ;
#17556=CIRCLE ( 'NONE', #109524, 0.06509327318403745899 ) ;
#17557=CIRCLE ( 'NONE', #122045, 0.06509327318403743123 ) ;
#17558=VERTEX_POINT ( 'NONE', #34454 ) ;
#17559=VECTOR ( 'NONE', #7887, 1000.000000000000000 ) ;
#17560=DIRECTION ( 'NONE',  ( 0.000000000000000000, -0.9999939076577903929, 0.003490651415223739937 ) ) ;
#17561=DIRECTION ( 'NONE',  ( -0.000000000000000000, 1.000000000000000000, -0.000000000000000000 ) ) ;
#17562=DIRECTION ( 'NONE',  ( -0.000000000000000000, -1.000000000000000000, -0.000000000000000000 ) ) ;
#17563=CONICAL_SURFACE ( 'NONE', #40601, 0.09999999999999982514, 0.003490658503988666988 ) ;
#17564=EDGE_LOOP ( 'NONE', ( #62073, #73258, #97491, #54644 ) ) ;
#17565=VERTEX_POINT ( 'NONE', #4300 ) ;
#17566=CARTESIAN_POINT ( 'NONE',  ( -9.600000000000006750, 12.50000000000000000, -0.6928203230275542523 ) ) ;
#17567=EDGE_LOOP ( 'NONE', ( #4599, #52117 ) ) ;
#17568=CARTESIAN_POINT ( 'NONE',  ( 8.099999999999923261, 2.500000000000000000, 4.676537180435972552 ) ) ;
#17569=FACE_BOUND ( 'NONE', #41180, .T. ) ;
#17570=ORIENTED_EDGE ( 'NONE', *, *, #64896, .F. ) ;
#17571=CARTESIAN_POINT ( 'NONE',  ( 4.149999999999938183, 12.50000000000000000, 5.802370205355744659 ) ) ;
#17572=ORIENTED_EDGE ( 'NONE', *, *, #68946, .F. ) ;
#17573=LINE ( 'NONE', #48338, #29478 ) ;
#17574=AXIS2_PLACEMENT_3D ( 'NONE', #59816, #68300, #88599 ) ;
#17575=DIRECTION ( 'NONE',  ( -0.000000000000000000, -1.000000000000000000, -0.000000000000000000 ) ) ;
#17576=CARTESIAN_POINT ( 'NONE',  ( 8.749999999999923617, 2.500000000000000000, -7.288010851410854585 ) ) ;
#17577=FACE_OUTER_BOUND ( 'NONE', #118449, .T. ) ;
#17578=DIRECTION ( 'NONE',  ( 0.000000000000000000, 0.000000000000000000, 1.000000000000000000 ) ) ;
#17579=AXIS2_PLACEMENT_3D ( 'NONE', #107124, #8283, #105854 ) ;
#17580=EDGE_LOOP ( 'NONE', ( #118211, #92492 ) ) ;
#17581=EDGE_CURVE ( 'NONE', #41455, #77736, #96391, .T. ) ;
#17582=ORIENTED_EDGE ( 'NONE', *, *, #25073, .T. ) ;
#17583=DIRECTION ( 'NONE',  ( 0.000000000000000000, -0.9999939076577903929, 0.003490651415223739937 ) ) ;
#17584=DIRECTION ( 'NONE',  ( 0.000000000000000000, 0.000000000000000000, -1.000000000000000000 ) ) ;
#17585=CARTESIAN_POINT ( 'NONE',  ( -1.250000000000001554, 12.50000000000000000, 2.099970236277060032 ) ) ;
#17586=ORIENTED_EDGE ( 'NONE', *, *, #96807, .F. ) ;
#17587=VERTEX_POINT ( 'NONE', #55997 ) ;
#17588=ORIENTED_EDGE ( 'NONE', *, *, #74964, .T. ) ;
#17589=FACE_OUTER_BOUND ( 'NONE', #55034, .T. ) ;
#17590=AXIS2_PLACEMENT_3D ( 'NONE', #76645, #109145, #19485 ) ;
#17591=FACE_OUTER_BOUND ( 'NONE', #31639, .T. ) ;
#17592=EDGE_CURVE ( 'NONE', #27692, #66554, #58761, .T. ) ;
#17593=CONICAL_SURFACE ( 'NONE', #19663, 0.1000000000000002554, 0.003490658503988666988 ) ;
#17594=CARTESIAN_POINT ( 'NONE',  ( -4.400000000000025224, 12.50000000000000000, 0.3464101615137735735 ) ) ;
#17596=LINE ( 'NONE', #67318, #41139 ) ;
#17597=DIRECTION ( 'NONE',  ( -0.000000000000000000, -1.000000000000000000, -0.000000000000000000 ) ) ;
#17598=CARTESIAN_POINT ( 'NONE',  ( -2.900000000000029221, 12.50000000000000000, -4.265033745738164406 ) ) ;
#17599=DIRECTION ( 'NONE',  ( -0.000000000000000000, -1.000000000000000000, -0.000000000000000000 ) ) ;
#17600=DIRECTION ( 'NONE',  ( 0.000000000000000000, 0.000000000000000000, 1.000000000000000000 ) ) ;
#17601=ADVANCED_FACE ( 'NONE', ( #25240 ), #65086, .T. ) ;
#17602=EDGE_CURVE ( 'NONE', #120216, #87169, #114915, .T. ) ;
#17603=CARTESIAN_POINT ( 'NONE',  ( 12.49999999999990052, 12.50000000000000000, 0.6928203230275494784 ) ) ;
#17604=EDGE_LOOP ( 'NONE', ( #25085, #28564 ) ) ;
#17605=EDGE_LOOP ( 'NONE', ( #35249, #107748 ) ) ;
#17606=AXIS2_PLACEMENT_3D ( 'NONE', #78869, #66440, #56604 ) ;
#17607=EDGE_CURVE ( 'NONE', #89288, #72494, #85923, .T. ) ;
#17608=FACE_OUTER_BOUND ( 'NONE', #75984, .T. ) ;
#17609=ORIENTED_EDGE ( 'NONE', *, *, #114046, .F. ) ;
#17610=ORIENTED_EDGE ( 'NONE', *, *, #60221, .T. ) ;
#17611=ADVANCED_FACE ( 'NONE', ( #103828 ), #14138, .T. ) ;
#17612=DIRECTION ( 'NONE',  ( -4.274815082592931898E-19, -0.9999939076577903929, -0.003490651415223739937 ) ) ;
#17613=DIRECTION ( 'NONE',  ( 0.000000000000000000, 0.000000000000000000, 1.000000000000000000 ) ) ;
#17614=DIRECTION ( 'NONE',  ( 0.000000000000000000, 0.000000000000000000, 1.000000000000000000 ) ) ;
#17615=FACE_OUTER_BOUND ( 'NONE', #114064, .T. ) ;
#17616=DIRECTION ( 'NONE',  ( -4.274815082592931898E-19, -0.9999939076577903929, -0.003490651415223739937 ) ) ;
#17617=AXIS2_PLACEMENT_3D ( 'NONE', #115892, #116533, #63584 ) ;
#17618=LINE ( 'NONE', #35983, #126320 ) ;
#17619=CONICAL_SURFACE ( 'NONE', #42699, 0.09999999999999982514, 0.003490658503988666988 ) ;
#17620=DIRECTION ( 'NONE',  ( 0.000000000000000000, -0.9999939076577903929, 0.003490651415223739937 ) ) ;
#17621=EDGE_LOOP ( 'NONE', ( #15190, #72563 ) ) ;
#17622=DIRECTION ( 'NONE',  ( 0.000000000000000000, 0.000000000000000000, 1.000000000000000000 ) ) ;
#17623=AXIS2_PLACEMENT_3D ( 'NONE', #44616, #65536, #123185 ) ;
#17624=AXIS2_PLACEMENT_3D ( 'NONE', #94636, #14142, #54085 ) ;
#17625=DIRECTION ( 'NONE',  ( 0.000000000000000000, 0.000000000000000000, 1.000000000000000000 ) ) ;
#17626=EDGE_LOOP ( 'NONE', ( #57369, #41175 ) ) ;
#17627=ADVANCED_FACE ( 'NONE', ( #4959 ), #42128, .T. ) ;
#17628=ORIENTED_EDGE ( 'NONE', *, *, #15718, .F. ) ;
#17629=VERTEX_POINT ( 'NONE', #15419 ) ;
#17630=ORIENTED_EDGE ( 'NONE', *, *, #52449, .T. ) ;
#17631=DIRECTION ( 'NONE',  ( 0.000000000000000000, 1.000000000000000000, 0.000000000000000000 ) ) ;
#17632=CARTESIAN_POINT ( 'NONE',  ( 7.899999999999924860, 2.500000000000000000, -5.022947341949754119 ) ) ;
#17634=CARTESIAN_POINT ( 'NONE',  ( -9.550000000000006040, 2.500000000000000000, 2.165063509461097713 ) ) ;
#17635=EDGE_CURVE ( 'NONE', #5027, #27825, #79680, .T. ) ;
#17636=CARTESIAN_POINT ( 'NONE',  ( -9.350000000000006750, 12.50000000000000000, 1.883746621131358934 ) ) ;
#17637=AXIS2_PLACEMENT_3D ( 'NONE', #70753, #61597, #1999 ) ;
#17638=AXIS2_PLACEMENT_3D ( 'NONE', #106499, #67181, #96033 ) ;
#17639=CARTESIAN_POINT ( 'NONE',  ( -2.300000000000032685, 2.500000000000000000, -4.676537180435978769 ) ) ;
#17640=ORIENTED_EDGE ( 'NONE', *, *, #120342, .T. ) ;
#17641=CONICAL_SURFACE ( 'NONE', #19717, 0.09999999999999982514, 0.003490658503988666988 ) ;
#17642=DIRECTION ( 'NONE',  ( 0.000000000000000000, 0.000000000000000000, -1.000000000000000000 ) ) ;
#17643=EDGE_CURVE ( 'NONE', #89461, #74255, #75631, .T. ) ;
#17644=DIRECTION ( 'NONE',  ( 0.000000000000000000, -0.000000000000000000, 1.000000000000000000 ) ) ;
#17645=EDGE_LOOP ( 'NONE', ( #97776, #81373 ) ) ;
#17647=CIRCLE ( 'NONE', #51127, 0.09999999999999982514 ) ;
#17648=ORIENTED_EDGE ( 'NONE', *, *, #39741, .T. ) ;
#17649=ORIENTED_EDGE ( 'NONE', *, *, #7406, .F. ) ;
#17650=PLANE ( 'NONE',  #124188 ) ;
#17651=EDGE_CURVE ( 'NONE', #38892, #97893, #42035, .T. ) ;
#17652=EDGE_CURVE ( 'NONE', #41301, #82923, #35101, .T. ) ;
#17653=EDGE_CURVE ( 'NONE', #58662, #38209, #46232, .T. ) ;
#17654=DIRECTION ( 'NONE',  ( 0.000000000000000000, 0.000000000000000000, 1.000000000000000000 ) ) ;
#17655=CIRCLE ( 'NONE', #82442, 0.06509327318403745899 ) ;
#17656=AXIS2_PLACEMENT_3D ( 'NONE', #75195, #115089, #25427 ) ;
#17657=ADVANCED_FACE ( 'NONE', ( #126023 ), #56676, .T. ) ;
#17658=CIRCLE ( 'NONE', #113825, 0.1000000000000002554 ) ;
#17659=EDGE_LOOP ( 'NONE', ( #120921, #66177, #109760, #64649 ) ) ;
#17660=DIRECTION ( 'NONE',  ( 0.000000000000000000, 0.000000000000000000, 1.000000000000000000 ) ) ;
#17661=PLANE ( 'NONE',  #43410 ) ;
#17662=PLANE ( 'NONE',  #19056 ) ;
#17663=FACE_OUTER_BOUND ( 'NONE', #95038, .T. ) ;
#17664=EDGE_CURVE ( 'NONE', #101480, #85870, #23238, .T. ) ;
#17665=VERTEX_POINT ( 'NONE', #6877 ) ;
#17666=EDGE_CURVE ( 'NONE', #122449, #34079, #59254, .T. ) ;
#17667=DIRECTION ( 'NONE',  ( 0.000000000000000000, 1.000000000000000000, 0.000000000000000000 ) ) ;
#17668=ORIENTED_EDGE ( 'NONE', *, *, #13919, .T. ) ;
#17669=ORIENTED_EDGE ( 'NONE', *, *, #31691, .T. ) ;
#17670=CARTESIAN_POINT ( 'NONE',  ( 11.44999999999991047, 2.500000000000000000, -2.411473670974877859 ) ) ;
#17671=DIRECTION ( 'NONE',  ( 0.000000000000000000, 0.000000000000000000, -1.000000000000000000 ) ) ;
#17672=FACE_BOUND ( 'NONE', #28304, .T. ) ;
#17673=CARTESIAN_POINT ( 'NONE',  ( 17.50000000000000000, 2.500000000000000000, 4.000000000000000888 ) ) ;
#17674=CONICAL_SURFACE ( 'NONE', #34428, 0.1000000000000002554, 0.003490658503988666988 ) ;
#17675=CARTESIAN_POINT ( 'NONE',  ( -9.150000000000005684, 2.500000000000000000, 7.188010851410848723 ) ) ;
#17676=DIRECTION ( 'NONE',  ( -0.000000000000000000, -1.000000000000000000, -0.000000000000000000 ) ) ;
#17677=ORIENTED_EDGE ( 'NONE', *, *, #4776, .T. ) ;
#17678=LINE ( 'NONE', #39302, #106974 ) ;
#17679=CARTESIAN_POINT ( 'NONE',  ( 7.899999999999924860, 2.500000000000000000, -3.737306695894649700 ) ) ;
#17680=ADVANCED_FACE ( 'NONE', ( #78893 ), #18008, .T. ) ;
#17681=CARTESIAN_POINT ( 'NONE',  ( 4.599999999999938360, 2.500000000000000000, -0.6928203230275541413 ) ) ;
#17682=CARTESIAN_POINT ( 'NONE',  ( -5.400000000000019895, 12.50000000000000000, -2.276824562219559311E-15 ) ) ;
#17683=ORIENTED_EDGE ( 'NONE', *, *, #64746, .F. ) ;
#17684=VECTOR ( 'NONE', #114946, 1000.000000000000000 ) ;
#17685=CIRCLE ( 'NONE', #28166, 0.1000000000000002554 ) ;
#17686=CARTESIAN_POINT ( 'NONE',  ( -8.950000000000009948, 12.50000000000000000, -6.841600689897072485 ) ) ;
#17687=CARTESIAN_POINT ( 'NONE',  ( 11.84999999999990727, 12.50000000000000000, -2.446380397790840266 ) ) ;
#17688=ORIENTED_EDGE ( 'NONE', *, *, #117204, .T. ) ;
#17689=DIRECTION ( 'NONE',  ( 0.000000000000000000, 0.000000000000000000, -1.000000000000000000 ) ) ;
#17690=FACE_OUTER_BOUND ( 'NONE', #127939, .T. ) ;
#17691=FACE_BOUND ( 'NONE', #41565, .T. ) ;
#17692=DIRECTION ( 'NONE',  ( -0.000000000000000000, 1.000000000000000000, -0.000000000000000000 ) ) ;
#17693=ORIENTED_EDGE ( 'NONE', *, *, #32175, .F. ) ;
#17694=DIRECTION ( 'NONE',  ( 0.000000000000000000, 1.000000000000000000, 0.000000000000000000 ) ) ;
#17695=VECTOR ( 'NONE', #98845, 1000.000000000000000 ) ;
#17696=ORIENTED_EDGE ( 'NONE', *, *, #101543, .F. ) ;
#17697=ORIENTED_EDGE ( 'NONE', *, *, #30231, .F. ) ;
#17698=CARTESIAN_POINT ( 'NONE',  ( 20.80940928220359609, 0.7000174339601031859, -4.161255421338316829 ) ) ;
#17700=VERTEX_POINT ( 'NONE', #9491 ) ;
#17701=DIRECTION ( 'NONE',  ( 0.000000000000000000, -0.000000000000000000, 1.000000000000000000 ) ) ;
#17702=CARTESIAN_POINT ( 'NONE',  ( -2.100000000000033840, 2.500000000000000000, 5.122947341949749323 ) ) ;
#17703=ADVANCED_FACE ( 'NONE', ( #48779 ), #21283, .T. ) ;
#17704=AXIS2_PLACEMENT_3D ( 'NONE', #7865, #77264, #29459 ) ;
#17705=AXIS2_PLACEMENT_3D ( 'NONE', #21728, #101576, #52461 ) ;
#17706=CIRCLE ( 'NONE', #17417, 0.1000000000000002554 ) ;
#17707=CARTESIAN_POINT ( 'NONE',  ( -4.119968255444916849E-14, 12.50000000000000000, 3.637306695894644726 ) ) ;
#17708=ORIENTED_EDGE ( 'NONE', *, *, #92729, .T. ) ;
#17710=CARTESIAN_POINT ( 'NONE',  ( -3.100000000000028511, 2.500000000000000000, -4.676537180435977881 ) ) ;
#17711=CARTESIAN_POINT ( 'NONE',  ( -10.00000000000000711, 2.500000000000000000, -3.537306695894645969 ) ) ;
#17712=CARTESIAN_POINT ( 'NONE',  ( 18.45986578164202996, -0.7763536479255006562, -4.045836815165628764 ) ) ;
#17713=ORIENTED_EDGE ( 'NONE', *, *, #3450, .F. ) ;
#17714=CARTESIAN_POINT ( 'NONE',  ( 11.64999999999990621, 12.50000000000000000, 6.495190528383297135 ) ) ;
#17715=VERTEX_POINT ( 'NONE', #7540 ) ;
#17716=DIRECTION ( 'NONE',  ( -0.000000000000000000, -1.000000000000000000, -0.000000000000000000 ) ) ;
#17717=VERTEX_POINT ( 'NONE', #108953 ) ;
#17718=CARTESIAN_POINT ( 'NONE',  ( 14.99999999999989342, 2.500000000000000000, -0.7928203230275542301 ) ) ;
#17719=CARTESIAN_POINT ( 'NONE',  ( 87.49999999999998579, -5.708722954879575262, 4.899943752027914989 ) ) ;
#17720=DIRECTION ( 'NONE',  ( -0.000000000000000000, 1.000000000000000000, -0.000000000000000000 ) ) ;
#17721=AXIS2_PLACEMENT_3D ( 'NONE', #77199, #37912, #105369 ) ;
#17722=DIRECTION ( 'NONE',  ( 0.000000000000000000, -0.000000000000000000, 1.000000000000000000 ) ) ;
#17723=ORIENTED_EDGE ( 'NONE', *, *, #9371, .T. ) ;
#17724=VECTOR ( 'NONE', #41655, 1000.000000000000000 ) ;
#17725=CARTESIAN_POINT ( 'NONE',  ( 3.099999999999945466, 2.500000000000000000, -3.983716857408426293 ) ) ;
#17726=CARTESIAN_POINT ( 'NONE',  ( -11.25000000000000178, 2.500000000000000000, -1.372243186433546036 ) ) ;
#17727=AXIS2_PLACEMENT_3D ( 'NONE', #9423, #8752, #99746 ) ;
#17728=VECTOR ( 'NONE', #78938, 1000.000000000000000 ) ;
#17729=CARTESIAN_POINT ( 'NONE',  ( -0.8000000000000376810, 2.500000000000000000, -4.330127018922201643 ) ) ;
#17730=DIRECTION ( 'NONE',  ( 0.000000000000000000, 1.000000000000000000, 0.000000000000000000 ) ) ;
#17731=CARTESIAN_POINT ( 'NONE',  ( 4.149999999999938183, 2.500000000000000000, 7.188010851410848723 ) ) ;
#17732=VECTOR ( 'NONE', #81391, 1000.000000000000000 ) ;
#17733=ORIENTED_EDGE ( 'NONE', *, *, #33326, .F. ) ;
#17734=VECTOR ( 'NONE', #124317, 1000.000000000000000 ) ;
#17735=VERTEX_POINT ( 'NONE', #19958 ) ;
#17736=VECTOR ( 'NONE', #20531, 1000.000000000000000 ) ;
#17737=DIRECTION ( 'NONE',  ( -0.000000000000000000, 1.000000000000000000, -0.000000000000000000 ) ) ;
#17738=ORIENTED_EDGE ( 'NONE', *, *, #63174, .F. ) ;
#17739=B_SPLINE_CURVE_WITH_KNOTS ( 'NONE', 3,
 ( #126101, #35797, #84238, #55437, #5032, #86822, #86158, #46251, #37098, #35173 ),
 .UNSPECIFIED., .F., .F.,
 ( 4, 2, 2, 2, 4 ),
 ( -0.0001133383185230014501, 0.01648989986483693007, 0.03309313804819685734, 0.04969637623155678807, 0.06629961441491671881 ),
 .UNSPECIFIED. ) ;
#17740=LINE ( 'NONE', #57689, #17979 ) ;
#17741=VECTOR ( 'NONE', #6354, 1000.000000000000000 ) ;
#17742=ORIENTED_EDGE ( 'NONE', *, *, #25479, .F. ) ;
#17743=ORIENTED_EDGE ( 'NONE', *, *, #2256, .F. ) ;
#17744=ORIENTED_EDGE ( 'NONE', *, *, #97126, .T. ) ;
#17745=CARTESIAN_POINT ( 'NONE',  ( -9.600000000000006750, 12.50000000000000000, 0.6277270498435120194 ) ) ;
#17746=AXIS2_PLACEMENT_3D ( 'NONE', #56719, #18752, #58052 ) ;
#17747=CARTESIAN_POINT ( 'NONE',  ( 8.749999999999920064, 12.50000000000000000, -2.922977105672691422 ) ) ;
#17748=ADVANCED_FACE ( 'NONE', ( #78243 ), #31766, .T. ) ;
#17749=DIRECTION ( 'NONE',  ( 0.000000000000000000, 1.000000000000000000, 0.000000000000000000 ) ) ;
#17750=CARTESIAN_POINT ( 'NONE',  ( -6.450000000000014388, 2.500000000000000000, 1.718653347947321386 ) ) ;
#17751=PLANE ( 'NONE',  #60630 ) ;
#17752=AXIS2_PLACEMENT_3D ( 'NONE', #1056, #109731, #69804 ) ;
#17753=CARTESIAN_POINT ( 'NONE',  ( -5.650000000000019895, 12.50000000000000000, 2.576566944158910744 ) ) ;
#17754=CARTESIAN_POINT ( 'NONE',  ( -10.20000000000000462, 2.500000000000000000, 4.776537180435972196 ) ) ;
#17755=EDGE_CURVE ( 'NONE', #38783, #5075, #50519, .T. ) ;
#17756=ORIENTED_EDGE ( 'NONE', *, *, #62244, .T. ) ;
#17757=EDGE_CURVE ( 'NONE', #64023, #98238, #29147, .T. ) ;
#17758=DIRECTION ( 'NONE',  ( 0.000000000000000000, 1.000000000000000000, 0.000000000000000000 ) ) ;
#17759=ORIENTED_EDGE ( 'NONE', *, *, #27403, .T. ) ;
#17760=ORIENTED_EDGE ( 'NONE', *, *, #49770, .F. ) ;
#17761=VERTEX_POINT ( 'NONE', #59903 ) ;
#17762=EDGE_LOOP ( 'NONE', ( #32980, #101069 ) ) ;
#17763=EDGE_CURVE ( 'NONE', #64667, #104068, #69042, .T. ) ;
#17764=CARTESIAN_POINT ( 'NONE',  ( -10.84999999999999964, 12.50000000000000000, 5.802370205355744659 ) ) ;
#17765=ADVANCED_FACE ( 'NONE', ( #107022 ), #33803, .T. ) ;
#17766=EDGE_CURVE ( 'NONE', #114247, #10596, #18658, .T. ) ;
#17767=ORIENTED_EDGE ( 'NONE', *, *, #96524, .F. ) ;
#17768=ORIENTED_EDGE ( 'NONE', *, *, #62106, .T. ) ;
#17769=EDGE_CURVE ( 'NONE', #1435, #103138, #115347, .T. ) ;
#17770=CIRCLE ( 'NONE', #32483, 0.1000000000000002554 ) ;
#17771=DIRECTION ( 'NONE',  ( 0.000000000000000000, 0.000000000000000000, 1.000000000000000000 ) ) ;
#17772=DIRECTION ( 'NONE',  ( -0.000000000000000000, 1.000000000000000000, -0.000000000000000000 ) ) ;
#17773=DIRECTION ( 'NONE',  ( 0.000000000000000000, 1.000000000000000000, 0.000000000000000000 ) ) ;
#17774=FACE_OUTER_BOUND ( 'NONE', #119639, .T. ) ;
#17775=DIRECTION ( 'NONE',  ( 0.000000000000000000, 0.000000000000000000, 1.000000000000000000 ) ) ;
#17776=VERTEX_POINT ( 'NONE', #10137 ) ;
#17777=CARTESIAN_POINT ( 'NONE',  ( -4.294451507785425339E-14, 12.50000000000000000, 4.957854068765711553 ) ) ;
#17778=VECTOR ( 'NONE', #120126, 1000.000000000000000 ) ;
#17779=CIRCLE ( 'NONE', #38654, 0.06509327318403745899 ) ;
#17780=ORIENTED_EDGE ( 'NONE', *, *, #124543, .F. ) ;
#17781=CARTESIAN_POINT ( 'NONE',  ( -12.29999999999999538, 2.500000000000000000, 4.776537180435972196 ) ) ;
#17783=CARTESIAN_POINT ( 'NONE',  ( 11.04999999999991189, 2.500000000000000000, -2.411473670974877859 ) ) ;
#17784=ORIENTED_EDGE ( 'NONE', *, *, #118962, .T. ) ;
#17785=EDGE_LOOP ( 'NONE', ( #28389, #21369, #64760, #68131 ) ) ;
#17786=DIRECTION ( 'NONE',  ( 0.000000000000000000, 0.000000000000000000, 1.000000000000000000 ) ) ;
#17787=DIRECTION ( 'NONE',  ( 0.000000000000000000, 0.000000000000000000, -1.000000000000000000 ) ) ;
#17788=CIRCLE ( 'NONE', #32498, 0.1000000000000002554 ) ;
#17789=DIRECTION ( 'NONE',  ( -0.000000000000000000, 1.000000000000000000, -0.000000000000000000 ) ) ;
#17790=CARTESIAN_POINT ( 'NONE',  ( -13.34999999999999076, 12.50000000000000000, -2.857883832488651521 ) ) ;
#17791=CIRCLE ( 'NONE', #45005, 0.1000000000000000472 ) ;
#17792=CARTESIAN_POINT ( 'NONE',  ( 13.34999999999990017, 12.50000000000000000, 2.857883832488649301 ) ) ;
#17793=EDGE_LOOP ( 'NONE', ( #122567, #125241 ) ) ;
#17794=DIRECTION ( 'NONE',  ( -4.274815082592931898E-19, -0.9999939076577903929, -0.003490651415223739937 ) ) ;
#17795=DIRECTION ( 'NONE',  ( -0.000000000000000000, 1.000000000000000000, -0.000000000000000000 ) ) ;
#17796=EDGE_CURVE ( 'NONE', #20424, #11168, #88017, .T. ) ;
#17797=CARTESIAN_POINT ( 'NONE',  ( 1.249999999999988454, 2.500000000000000000, 2.265063509461097357 ) ) ;
#17799=DIRECTION ( 'NONE',  ( 0.000000000000000000, 0.000000000000000000, 1.000000000000000000 ) ) ;
#17800=ORIENTED_EDGE ( 'NONE', *, *, #29308, .T. ) ;
#17801=AXIS2_PLACEMENT_3D ( 'NONE', #19991, #19320, #97889 ) ;
#17802=ORIENTED_EDGE ( 'NONE', *, *, #121783, .T. ) ;
#17803=EDGE_CURVE ( 'NONE', #5314, #125017, #76946, .T. ) ;
#17804=CARTESIAN_POINT ( 'NONE',  ( -2.700000000000030820, 12.50000000000000000, -3.918623584224389056 ) ) ;
#17805=EDGE_CURVE ( 'NONE', #69443, #112225, #104893, .T. ) ;
#17806=EDGE_CURVE ( 'NONE', #120000, #102762, #2386, .T. ) ;
#17807=VERTEX_POINT ( 'NONE', #37671 ) ;
#17808=CARTESIAN_POINT ( 'NONE',  ( -5.650000000000023448, 12.50000000000000000, -1.818653347947326138 ) ) ;
#17809=PLANE ( 'NONE',  #12496 ) ;
#17810=ADVANCED_FACE ( 'NONE', ( #57953 ), #19110, .T. ) ;
#17811=ORIENTED_EDGE ( 'NONE', *, *, #39272, .F. ) ;
#17813=DIRECTION ( 'NONE',  ( 0.000000000000000000, 1.000000000000000000, 0.000000000000000000 ) ) ;
#17814=ADVANCED_FACE ( 'NONE', ( #28491 ), #127969, .T. ) ;
#17815=DIRECTION ( 'NONE',  ( 0.000000000000000000, -0.000000000000000000, 1.000000000000000000 ) ) ;
#17816=CONICAL_SURFACE ( 'NONE', #34576, 0.1000000000000002554, 0.003490658503988666988 ) ;
#17817=FACE_OUTER_BOUND ( 'NONE', #101641, .T. ) ;
#17818=VERTEX_POINT ( 'NONE', #128648 ) ;
#17819=ADVANCED_FACE ( 'NONE', ( #40241 ), #80162, .T. ) ;
#17820=ADVANCED_FACE ( 'NONE', ( #122661 ), #92289, .T. ) ;
#17821=ADVANCED_FACE ( 'NONE', ( #91270 ), #72289, .T. ) ;
#17822=AXIS2_PLACEMENT_3D ( 'NONE', #81699, #73809, #72548 ) ;
#17823=CARTESIAN_POINT ( 'NONE',  ( -6.900000000000015454, 2.500000000000000000, 4.676537180435972552 ) ) ;
#17824=CARTESIAN_POINT ( 'NONE',  ( -3.350000000000028511, 2.500000000000000000, -1.472243186433550122 ) ) ;
#17825=CIRCLE ( 'NONE', #99316, 0.06509327318403745899 ) ;
#17826=EDGE_LOOP ( 'NONE', ( #123734, #69264, #42843, #37200 ) ) ;
#17827=AXIS2_PLACEMENT_3D ( 'NONE', #76678, #57016, #56378 ) ;
#17828=DIRECTION ( 'NONE',  ( 0.000000000000000000, 0.000000000000000000, 1.000000000000000000 ) ) ;
#17829=CARTESIAN_POINT ( 'NONE',  ( 0.5999999999999551248, 2.500000000000000000, -4.676537180435978769 ) ) ;
#17830=EDGE_CURVE ( 'NONE', #78336, #22216, #46317, .T. ) ;
#17831=DIRECTION ( 'NONE',  ( -0.000000000000000000, 1.000000000000000000, -0.000000000000000000 ) ) ;
#17832=AXIS2_PLACEMENT_3D ( 'NONE', #38073, #126461, #78657 ) ;
#17833=AXIS2_PLACEMENT_3D ( 'NONE', #87600, #127541, #59473 ) ;
#17834=EDGE_LOOP ( 'NONE', ( #82588, #117974, #101761, #49621 ) ) ;
#17835=AXIS2_PLACEMENT_3D ( 'NONE', #122596, #102944, #32946 ) ;
#17836=DIRECTION ( 'NONE',  ( 0.000000000000000000, 0.000000000000000000, 1.000000000000000000 ) ) ;
#17837=AXIS2_PLACEMENT_3D ( 'NONE', #57271, #55338, #85434 ) ;
#17838=ORIENTED_EDGE ( 'NONE', *, *, #26404, .T. ) ;
#17839=PLANE ( 'NONE',  #64726 ) ;
#17840=CARTESIAN_POINT ( 'NONE',  ( -12.69999999999999396, 12.50000000000000000, 0.3464101615137776813 ) ) ;
#17841=CARTESIAN_POINT ( 'NONE',  ( -14.34999999999998543, 12.50000000000000000, -2.446380397790838046 ) ) ;
#17842=ORIENTED_EDGE ( 'NONE', *, *, #30634, .T. ) ;
#17843=AXIS2_PLACEMENT_3D ( 'NONE', #43579, #86033, #125970 ) ;
#17844=VECTOR ( 'NONE', #62972, 1000.000000000000000 ) ;
#17845=CARTESIAN_POINT ( 'NONE',  ( 15.39999999999989200, 2.500000000000000000, 0.5928203230275495006 ) ) ;
#17846=AXIS2_PLACEMENT_3D ( 'NONE', #70892, #51271, #50593 ) ;
#17847=DIRECTION ( 'NONE',  ( -0.000000000000000000, 1.000000000000000000, -0.000000000000000000 ) ) ;
#17848=ORIENTED_EDGE ( 'NONE', *, *, #40430, .F. ) ;
#17849=DIRECTION ( 'NONE',  ( 0.000000000000000000, 1.000000000000000000, 0.000000000000000000 ) ) ;
#17850=ORIENTED_EDGE ( 'NONE', *, *, #42664, .T. ) ;
#17851=PLANE ( 'NONE',  #114225 ) ;
#17852=EDGE_LOOP ( 'NONE', ( #98182, #31989 ) ) ;
#17853=CARTESIAN_POINT ( 'NONE',  ( 0.000000000000000000, 1.500000000000000000, 9.000000000000001776 ) ) ;
#17854=DIRECTION ( 'NONE',  ( 0.000000000000000000, 0.000000000000000000, 1.000000000000000000 ) ) ;
#17856=ORIENTED_EDGE ( 'NONE', *, *, #27853, .F. ) ;
#17857=DIRECTION ( 'NONE',  ( 0.000000000000000000, 0.000000000000000000, 1.000000000000000000 ) ) ;
#17858=CARTESIAN_POINT ( 'NONE',  ( -4.350000000000027178, 12.50000000000000000, -6.776507416713039689 ) ) ;
#17859=AXIS2_PLACEMENT_3D ( 'NONE', #79872, #39957, #30793 ) ;
#17860=VERTEX_POINT ( 'NONE', #22549 ) ;
#17861=CARTESIAN_POINT ( 'NONE',  ( 4.349999999999939249, 2.500000000000000000, 2.511473670974873507 ) ) ;
#17862=FACE_OUTER_BOUND ( 'NONE', #48028, .T. ) ;
#17863=EDGE_CURVE ( 'NONE', #126669, #115818, #71442, .T. ) ;
#17864=DIRECTION ( 'NONE',  ( 0.000000000000000000, 1.000000000000000000, 0.000000000000000000 ) ) ;
#17865=DIRECTION ( 'NONE',  ( 0.000000000000000000, 1.000000000000000000, 0.000000000000000000 ) ) ;
#17866=CARTESIAN_POINT ( 'NONE',  ( -9.550000000000006040, 2.500000000000000000, 2.065063509461097624 ) ) ;
#17867=CIRCLE ( 'NONE', #53394, 0.06509327318403745899 ) ;
#17868=CARTESIAN_POINT ( 'NONE',  ( 8.949999999999915801, 12.50000000000000000, 6.906693963081109722 ) ) ;
#17869=CIRCLE ( 'NONE', #22109, 0.1000000000000002554 ) ;
#17870=AXIS2_PLACEMENT_3D ( 'NONE', #104472, #36400, #56007 ) ;
#17871=ORIENTED_EDGE ( 'NONE', *, *, #29173, .F. ) ;
#17872=ORIENTED_EDGE ( 'NONE', *, *, #14243, .T. ) ;
#17873=VERTEX_POINT ( 'NONE', #20601 ) ;
#17874=EDGE_LOOP ( 'NONE', ( #101890, #101951, #78743, #126517 ) ) ;
#17875=CARTESIAN_POINT ( 'NONE',  ( -2.900000000000029221, 12.50000000000000000, -4.395220292106239768 ) ) ;
#17876=DIRECTION ( 'NONE',  ( 0.000000000000000000, 0.000000000000000000, 1.000000000000000000 ) ) ;
#17877=DIRECTION ( 'NONE',  ( -0.000000000000000000, -1.000000000000000000, -0.000000000000000000 ) ) ;
#17878=ORIENTED_EDGE ( 'NONE', *, *, #13674, .T. ) ;
#17879=ADVANCED_FACE ( 'NONE', ( #51367 ), #113214, .T. ) ;
#17880=FACE_BOUND ( 'NONE', #54738, .T. ) ;
#17881=EDGE_LOOP ( 'NONE', ( #27967, #1167, #64929, #58686 ) ) ;
#17882=DIRECTION ( 'NONE',  ( 0.000000000000000000, 1.000000000000000000, 0.000000000000000000 ) ) ;
#17883=CARTESIAN_POINT ( 'NONE',  ( -8.150000000000012790, 12.50000000000000000, 1.753560074763284016 ) ) ;
#17884=VECTOR ( 'NONE', #49099, 1000.000000000000000 ) ;
#17885=DIRECTION ( 'NONE',  ( 0.000000000000000000, 0.000000000000000000, -1.000000000000000000 ) ) ;
#17886=CARTESIAN_POINT ( 'NONE',  ( -7.500000000000016875, 2.500000000000000000, -3.537306695894649966 ) ) ;
#17887=AXIS2_PLACEMENT_3D ( 'NONE', #112396, #43036, #50256 ) ;
#17888=FACE_OUTER_BOUND ( 'NONE', #18005, .T. ) ;
#17889=FACE_OUTER_BOUND ( 'NONE', #87233, .T. ) ;
#17890=FACE_OUTER_BOUND ( 'NONE', #59828, .T. ) ;
#17891=DIRECTION ( 'NONE',  ( -0.000000000000000000, 1.000000000000000000, -0.000000000000000000 ) ) ;
#17892=DIRECTION ( 'NONE',  ( -0.000000000000000000, -1.000000000000000000, -0.000000000000000000 ) ) ;
#17893=DIRECTION ( 'NONE',  ( 0.000000000000000000, -0.000000000000000000, 1.000000000000000000 ) ) ;
#17894=AXIS2_PLACEMENT_3D ( 'NONE', #801, #99664, #87879 ) ;
#17895=EDGE_LOOP ( 'NONE', ( #34435, #91252 ) ) ;
#17896=ORIENTED_EDGE ( 'NONE', *, *, #37823, .F. ) ;
#17897=AXIS2_PLACEMENT_3D ( 'NONE', #98372, #8693, #48651 ) ;
#17898=ORIENTED_EDGE ( 'NONE', *, *, #36439, .F. ) ;
#17899=VERTEX_POINT ( 'NONE', #63095 ) ;
#17900=CARTESIAN_POINT ( 'NONE',  ( 17.50000000000000000, -2.500000000000000000, -2.922290670087884124 ) ) ;
#17901=CARTESIAN_POINT ( 'NONE',  ( 0.6499999999999561684, 2.500000000000000000, 2.511473670974873507 ) ) ;
#17902=ORIENTED_EDGE ( 'NONE', *, *, #27216, .F. ) ;
#17903=ORIENTED_EDGE ( 'NONE', *, *, #107218, .T. ) ;
#17904=EDGE_LOOP ( 'NONE', ( #109604, #64135 ) ) ;
#17905=CARTESIAN_POINT ( 'NONE',  ( 1.249999999999953815, 12.50000000000000000, -2.857883832488653741 ) ) ;
#17907=FACE_OUTER_BOUND ( 'NONE', #47444, .T. ) ;
#17908=CARTESIAN_POINT ( 'NONE',  ( -10.00000000000000355, 12.50000000000000000, -0.6928203230275541413 ) ) ;
#17909=DIRECTION ( 'NONE',  ( 0.000000000000000000, 0.000000000000000000, 1.000000000000000000 ) ) ;
#17910=FACE_OUTER_BOUND ( 'NONE', #62186, .T. ) ;
#17912=AXIS2_PLACEMENT_3D ( 'NONE', #128887, #39219, #27413 ) ;
#17913=EDGE_LOOP ( 'NONE', ( #49271, #123797 ) ) ;
#17914=EDGE_CURVE ( 'NONE', #54140, #96322, #56759, .T. ) ;
#17915=CARTESIAN_POINT ( 'NONE',  ( 7.899999999999921307, 12.50000000000000000, -0.06509327318403980434 ) ) ;
#17916=ORIENTED_EDGE ( 'NONE', *, *, #63030, .T. ) ;
#17917=CIRCLE ( 'NONE', #91079, 0.1000000000000002554 ) ;
#17918=EDGE_LOOP ( 'NONE', ( #119085, #128669 ) ) ;
#17919=VERTEX_POINT ( 'NONE', #1586 ) ;
#17920=AXIS2_PLACEMENT_3D ( 'NONE', #82704, #122618, #73496 ) ;
#17921=EDGE_CURVE ( 'NONE', #11906, #45961, #123668, .T. ) ;
#17922=DIRECTION ( 'NONE',  ( 0.000000000000000000, -0.9999939076577903929, 0.003490651415223739937 ) ) ;
#17923=EDGE_CURVE ( 'NONE', #56262, #98108, #14996, .T. ) ;
#17925=EDGE_CURVE ( 'NONE', #80384, #114882, #88153, .T. ) ;
#17926=VERTEX_POINT ( 'NONE', #50697 ) ;
#17927=ADVANCED_FACE ( 'NONE', ( #952 ), #17033, .T. ) ;
#17928=EDGE_CURVE ( 'NONE', #15359, #6313, #53295, .T. ) ;
#17929=ORIENTED_EDGE ( 'NONE', *, *, #46398, .T. ) ;
#17930=CARTESIAN_POINT ( 'NONE',  ( -2.100000000000033396, 2.500000000000000000, -0.6928203230275542523 ) ) ;
#17931=DIRECTION ( 'NONE',  ( 0.000000000000000000, 0.000000000000000000, -1.000000000000000000 ) ) ;
#17932=DIRECTION ( 'NONE',  ( 0.000000000000000000, 0.000000000000000000, -1.000000000000000000 ) ) ;
#17933=CARTESIAN_POINT ( 'NONE',  ( 8.549999999999924327, 2.500000000000000000, -6.741600689897077281 ) ) ;
#17934=FACE_OUTER_BOUND ( 'NONE', #125302, .T. ) ;
#17935=EDGE_CURVE ( 'NONE', #48604, #10563, #52001, .T. ) ;
#17936=ORIENTED_EDGE ( 'NONE', *, *, #58141, .T. ) ;
#17937=DIRECTION ( 'NONE',  ( 0.000000000000000000, 1.000000000000000000, 0.000000000000000000 ) ) ;
#17938=EDGE_CURVE ( 'NONE', #26160, #64274, #110895, .T. ) ;
#17939=AXIS2_PLACEMENT_3D ( 'NONE', #77521, #48080, #117418 ) ;
#17940=VECTOR ( 'NONE', #68762, 1000.000000000000000 ) ;
#17941=EDGE_CURVE ( 'NONE', #22615, #116464, #81911, .T. ) ;
#17942=ORIENTED_EDGE ( 'NONE', *, *, #66101, .T. ) ;
#17943=FACE_OUTER_BOUND ( 'NONE', #53416, .T. ) ;
#17944=CIRCLE ( 'NONE', #109897, 0.06509327318403745899 ) ;
#17945=ORIENTED_EDGE ( 'NONE', *, *, #107795, .F. ) ;
#17947=CARTESIAN_POINT ( 'NONE',  ( -4.150000000000025224, 2.500000000000000000, 6.495190528383297135 ) ) ;
#17948=CONICAL_SURFACE ( 'NONE', #89053, 0.1000000000000002554, 0.003490658503988666988 ) ;
#17949=ORIENTED_EDGE ( 'NONE', *, *, #121327, .T. ) ;
#17950=DIRECTION ( 'NONE',  ( -0.000000000000000000, -1.000000000000000000, -0.000000000000000000 ) ) ;
#17951=CARTESIAN_POINT ( 'NONE',  ( -6.850000000000017408, 12.50000000000000000, -1.818653347947325916 ) ) ;
#17952=ORIENTED_EDGE ( 'NONE', *, *, #2514, .T. ) ;
#17953=DIRECTION ( 'NONE',  ( -0.000000000000000000, -1.000000000000000000, -0.000000000000000000 ) ) ;
#17955=EDGE_LOOP ( 'NONE', ( #47487, #76341 ) ) ;
#17956=CARTESIAN_POINT ( 'NONE',  ( 5.849999999999933031, 12.50000000000000000, -1.407149913249512663 ) ) ;
#17957=CARTESIAN_POINT ( 'NONE',  ( 10.19999999999991402, 2.500000000000000000, 0.4464101615137735513 ) ) ;
#17959=CONICAL_SURFACE ( 'NONE', #120376, 0.09999999999999982514, 0.003490658503988666988 ) ;
#17960=CARTESIAN_POINT ( 'NONE',  ( -11.24999999999999822, 12.50000000000000000, 1.472243186433545459 ) ) ;
#17961=CARTESIAN_POINT ( 'NONE',  ( 9.349999999999919709, 2.500000000000000000, 2.411473670974873862 ) ) ;
#17962=DIRECTION ( 'NONE',  ( -0.000000000000000000, 1.000000000000000000, -0.000000000000000000 ) ) ;
#17963=AXIS2_PLACEMENT_3D ( 'NONE', #100786, #122390, #51080 ) ;
#17964=VECTOR ( 'NONE', #2083, 1000.000000000000000 ) ;
#17965=VERTEX_POINT ( 'NONE', #91915 ) ;
#17966=DIRECTION ( 'NONE',  ( 0.000000000000000000, 0.000000000000000000, -1.000000000000000000 ) ) ;
#17967=DIRECTION ( 'NONE',  ( 0.000000000000000000, -0.000000000000000000, 1.000000000000000000 ) ) ;
#17968=AXIS2_PLACEMENT_3D ( 'NONE', #117820, #47826, #28175 ) ;
#17969=ORIENTED_EDGE ( 'NONE', *, *, #93580, .T. ) ;
#17970=DIRECTION ( 'NONE',  ( -0.000000000000000000, -1.000000000000000000, -0.000000000000000000 ) ) ;
#17971=FACE_OUTER_BOUND ( 'NONE', #28141, .T. ) ;
#17972=DIRECTION ( 'NONE',  ( 0.000000000000000000, 0.000000000000000000, 1.000000000000000000 ) ) ;
#17973=EDGE_CURVE ( 'NONE', #64554, #81253, #117398, .T. ) ;
#17974=DIRECTION ( 'NONE',  ( 0.000000000000000000, 1.000000000000000000, 0.000000000000000000 ) ) ;
#17975=DIRECTION ( 'NONE',  ( 0.000000000000000000, 0.000000000000000000, 1.000000000000000000 ) ) ;
#17976=ORIENTED_EDGE ( 'NONE', *, *, #113289, .F. ) ;
#17977=CONICAL_SURFACE ( 'NONE', #107863, 0.1000000000000002554, 0.003490658503988666988 ) ;
#17978=EDGE_CURVE ( 'NONE', #104697, #97467, #58947, .T. ) ;
#17979=VECTOR ( 'NONE', #68130, 1000.000000000000000 ) ;
#17980=VECTOR ( 'NONE', #74084, 1000.000000000000000 ) ;
#17981=ADVANCED_FACE ( 'NONE', ( #103681 ), #123939, .T. ) ;
#17982=DIRECTION ( 'NONE',  ( 0.000000000000000000, 0.000000000000000000, 1.000000000000000000 ) ) ;
#17983=DIRECTION ( 'NONE',  ( 0.000000000000000000, -0.000000000000000000, 1.000000000000000000 ) ) ;
#17984=EDGE_LOOP ( 'NONE', ( #98974, #120625, #78155, #58723 ) ) ;
#17986=DIRECTION ( 'NONE',  ( 0.000000000000000000, 0.000000000000000000, 1.000000000000000000 ) ) ;
#17987=ORIENTED_EDGE ( 'NONE', *, *, #125059, .F. ) ;
#17989=LINE ( 'NONE', #17324, #105205 ) ;
#17990=VERTEX_POINT ( 'NONE', #23825 ) ;
#17991=PLANE ( 'NONE',  #67464 ) ;
#17992=CARTESIAN_POINT ( 'NONE',  ( -11.89999999999999503, 2.500000000000000000, 3.883716857408420431 ) ) ;
#17993=CARTESIAN_POINT ( 'NONE',  ( 0.5999999999999547917, 12.50000000000000000, 4.048810130592458201 ) ) ;
#17994=EDGE_LOOP ( 'NONE', ( #30889, #24018, #13911, #69106 ) ) ;
#17995=FACE_OUTER_BOUND ( 'NONE', #20492, .T. ) ;
#17996=DIRECTION ( 'NONE',  ( -0.000000000000000000, 1.000000000000000000, -0.000000000000000000 ) ) ;
#17997=VERTEX_POINT ( 'NONE', #96246 ) ;
#17998=CARTESIAN_POINT ( 'NONE',  ( -8.150000000000012790, 12.50000000000000000, 1.883746621131358934 ) ) ;
#17999=CARTESIAN_POINT ( 'NONE',  ( -10.65000000000000213, 2.500000000000000000, 6.048780366869520364 ) ) ;
#18000=ADVANCED_FACE ( 'NONE', ( #47171 ), #75647, .T. ) ;
#18001=ORIENTED_EDGE ( 'NONE', *, *, #120243, .T. ) ;
#18002=AXIS2_PLACEMENT_3D ( 'NONE', #61044, #51255, #1473 ) ;
#18003=ORIENTED_EDGE ( 'NONE', *, *, #5688, .F. ) ;
#18004=CIRCLE ( 'NONE', #51479, 0.06509327318403745899 ) ;
#18005=EDGE_LOOP ( 'NONE', ( #22441, #25831 ) ) ;
#18006=DIRECTION ( 'NONE',  ( -0.000000000000000000, 1.000000000000000000, -0.000000000000000000 ) ) ;
#18007=CARTESIAN_POINT ( 'NONE',  ( 3.549999999999943867, 2.500000000000000000, -1.718653347947326049 ) ) ;
#18008=PLANE ( 'NONE',  #12848 ) ;
#18009=FACE_BOUND ( 'NONE', #122218, .T. ) ;
#18010=ORIENTED_EDGE ( 'NONE', *, *, #127728, .T. ) ;
#18011=CARTESIAN_POINT ( 'NONE',  ( 14.99999999999989164, 12.50000000000000000, 0.6928203230275494784 ) ) ;
#18012=DIRECTION ( 'NONE',  ( 0.000000000000000000, 0.000000000000000000, 1.000000000000000000 ) ) ;
#18013=VERTEX_POINT ( 'NONE', #7872 ) ;
#18014=AXIS2_PLACEMENT_3D ( 'NONE', #13457, #93323, #123412 ) ;
#18016=EDGE_CURVE ( 'NONE', #58128, #119493, #27617, .T. ) ;
#18017=CARTESIAN_POINT ( 'NONE',  ( 105.5000000000000142, 0.000000000000000000, 0.000000000000000000 ) ) ;
#18018=DIRECTION ( 'NONE',  ( -4.274815082592931898E-19, -0.9999939076577903929, -0.003490651415223739937 ) ) ;
#18019=DIRECTION ( 'NONE',  ( 0.000000000000000000, 0.000000000000000000, -1.000000000000000000 ) ) ;
#18020=FACE_OUTER_BOUND ( 'NONE', #56053, .T. ) ;
#18021=AXIS2_PLACEMENT_3D ( 'NONE', #5403, #83343, #52574 ) ;
#18022=AXIS2_PLACEMENT_3D ( 'NONE', #100908, #42675, #81289 ) ;
#18023=AXIS2_PLACEMENT_3D ( 'NONE', #81206, #58985, #91658 ) ;
#18024=EDGE_LOOP ( 'NONE', ( #112406, #20226, #60341, #20009 ) ) ;
#18025=ORIENTED_EDGE ( 'NONE', *, *, #73769, .F. ) ;
#18026=ORIENTED_EDGE ( 'NONE', *, *, #28281, .F. ) ;
#18027=ORIENTED_EDGE ( 'NONE', *, *, #39689, .F. ) ;
#18028=ORIENTED_EDGE ( 'NONE', *, *, #49861, .F. ) ;
#18029=FACE_OUTER_BOUND ( 'NONE', #31856, .T. ) ;
#18030=DIRECTION ( 'NONE',  ( 0.000000000000000000, 0.000000000000000000, 1.000000000000000000 ) ) ;
#18031=ORIENTED_EDGE ( 'NONE', *, *, #64476, .F. ) ;
#18032=ADVANCED_FACE ( 'NONE', ( #104313 ), #56861, .T. ) ;
#18033=FACE_BOUND ( 'NONE', #707, .T. ) ;
#18035=CARTESIAN_POINT ( 'NONE',  ( 12.09999999999990550, 12.50000000000000000, 4.330127018922196314 ) ) ;
#18036=DIRECTION ( 'NONE',  ( 0.000000000000000000, 1.000000000000000000, 0.000000000000000000 ) ) ;
#18037=LINE ( 'NONE', #39016, #88799 ) ;
#18038=DIRECTION ( 'NONE',  ( 0.000000000000000000, 1.000000000000000000, 0.000000000000000000 ) ) ;
#18039=CIRCLE ( 'NONE', #107936, 0.06509327318403745899 ) ;
#18040=ORIENTED_EDGE ( 'NONE', *, *, #62154, .F. ) ;
#18041=CARTESIAN_POINT ( 'NONE',  ( 11.89999999999990443, 12.50000000000000000, -0.3464101615137782364 ) ) ;
#18042=ORIENTED_EDGE ( 'NONE', *, *, #29335, .T. ) ;
#18043=VECTOR ( 'NONE', #64462, 1000.000000000000000 ) ;
#18044=ORIENTED_EDGE ( 'NONE', *, *, #74204, .F. ) ;
#18045=ORIENTED_EDGE ( 'NONE', *, *, #1695, .T. ) ;
#18046=DIRECTION ( 'NONE',  ( 0.000000000000000000, 0.000000000000000000, 1.000000000000000000 ) ) ;
#18047=LINE ( 'NONE', #77612, #8684 ) ;
#18048=CONICAL_SURFACE ( 'NONE', #7584, 0.09999999999999982514, 0.003490658503988666988 ) ;
#18049=DIRECTION ( 'NONE',  ( 0.000000000000000000, 0.000000000000000000, -1.000000000000000000 ) ) ;
#18050=ORIENTED_EDGE ( 'NONE', *, *, #39063, .T. ) ;
#18051=DIRECTION ( 'NONE',  ( 0.000000000000000000, 1.000000000000000000, 0.000000000000000000 ) ) ;
#18052=CIRCLE ( 'NONE', #64034, 0.06509327318403745899 ) ;
#18053=CIRCLE ( 'NONE', #126739, 0.06509327318403745899 ) ;
#18054=DIRECTION ( 'NONE',  ( 0.000000000000000000, 0.000000000000000000, 1.000000000000000000 ) ) ;
#18055=CIRCLE ( 'NONE', #103754, 0.1000000000000002554 ) ;
#18056=EDGE_CURVE ( 'NONE', #26032, #103454, #96572, .T. ) ;
#18057=FACE_OUTER_BOUND ( 'NONE', #68249, .T. ) ;
#18059=CARTESIAN_POINT ( 'NONE',  ( 8.149999999999920419, 2.500000000000000000, 6.841600689897072485 ) ) ;
#18060=FACE_OUTER_BOUND ( 'NONE', #13795, .T. ) ;
#18061=DIRECTION ( 'NONE',  ( 0.000000000000000000, 1.000000000000000000, 0.000000000000000000 ) ) ;
#18062=ORIENTED_EDGE ( 'NONE', *, *, #77491, .T. ) ;
#18063=CARTESIAN_POINT ( 'NONE',  ( -12.29999999999999716, 12.50000000000000000, 0.3464101615137776813 ) ) ;
#18064=AXIS2_PLACEMENT_3D ( 'NONE', #84009, #54540, #94471 ) ;
#18065=ADVANCED_FACE ( 'NONE', ( #74211 ), #125824, .T. ) ;
#18066=ORIENTED_EDGE ( 'NONE', *, *, #23690, .F. ) ;
#18067=CIRCLE ( 'NONE', #47329, 0.1000000000000002554 ) ;
#18068=ORIENTED_EDGE ( 'NONE', *, *, #52846, .T. ) ;
#18069=DIRECTION ( 'NONE',  ( 0.000000000000000000, -0.000000000000000000, 1.000000000000000000 ) ) ;
#18070=ADVANCED_FACE ( 'NONE', ( #14616 ), #68083, .T. ) ;
#18071=DIRECTION ( 'NONE',  ( -0.000000000000000000, -1.000000000000000000, -0.000000000000000000 ) ) ;
#18072=FACE_OUTER_BOUND ( 'NONE', #77690, .T. ) ;
#18073=EDGE_CURVE ( 'NONE', #94129, #104091, #87075, .T. ) ;
#18074=EDGE_CURVE ( 'NONE', #56898, #68530, #46409, .T. ) ;
#18075=EDGE_CURVE ( 'NONE', #106661, #105096, #29699, .T. ) ;
#18076=ORIENTED_EDGE ( 'NONE', *, *, #29086, .F. ) ;
#18077=EDGE_LOOP ( 'NONE', ( #30878, #19277, #47662, #3904 ) ) ;
#18078=CARTESIAN_POINT ( 'NONE',  ( 0.3999999999999628852, 12.50000000000000000, -0.7579135962115894909 ) ) ;
#18079=DIRECTION ( 'NONE',  ( 0.000000000000000000, 1.000000000000000000, 0.000000000000000000 ) ) ;
#18080=EDGE_CURVE ( 'NONE', #116825, #5168, #48577, .T. ) ;
#18081=DIRECTION ( 'NONE',  ( 0.000000000000000000, 1.000000000000000000, 0.000000000000000000 ) ) ;
#18082=ORIENTED_EDGE ( 'NONE', *, *, #42088, .F. ) ;
#18083=VERTEX_POINT ( 'NONE', #86434 ) ;
#18084=ADVANCED_FACE ( 'NONE', ( #108011 ), #92376, .T. ) ;
#18085=DIRECTION ( 'NONE',  ( 0.000000000000000000, 1.000000000000000000, 0.000000000000000000 ) ) ;
#18086=EDGE_CURVE ( 'NONE', #102089, #54506, #94534, .T. ) ;
#18087=ORIENTED_EDGE ( 'NONE', *, *, #125847, .F. ) ;
#18088=CARTESIAN_POINT ( 'NONE',  ( 9.549999999999918998, 2.500000000000000000, 2.165063509461097713 ) ) ;
#18089=EDGE_CURVE ( 'NONE', #17389, #19145, #27496, .T. ) ;
#18090=ADVANCED_FACE ( 'NONE', ( #17690 ), #19211, .T. ) ;
#18091=CARTESIAN_POINT ( 'NONE',  ( -0.8500000000000382805, 2.500000000000000000, -2.757883832488654097 ) ) ;
#18093=CARTESIAN_POINT ( 'NONE',  ( -2.100000000000034284, 2.500000000000000000, -4.430127018922202176 ) ) ;
#18094=DIRECTION ( 'NONE',  ( 0.000000000000000000, 0.000000000000000000, 1.000000000000000000 ) ) ;
#18095=DIRECTION ( 'NONE',  ( 0.000000000000000000, 0.000000000000000000, 1.000000000000000000 ) ) ;
#18096=DIRECTION ( 'NONE',  ( -4.274815082592931898E-19, -0.9999939076577903929, -0.003490651415223739937 ) ) ;
#18097=EDGE_CURVE ( 'NONE', #41716, #91777, #102834, .T. ) ;
#18098=VERTEX_POINT ( 'NONE', #38660 ) ;
#18099=CARTESIAN_POINT ( 'NONE',  ( 17.50000000000000000, -2.500000000000000000, 4.000000000000001776 ) ) ;
#18100=CONICAL_SURFACE ( 'NONE', #13892, 0.1000000000000002554, 0.003490658503988666988 ) ;
#18101=CONICAL_SURFACE ( 'NONE', #26436, 0.1000000000000000472, 0.003490658503988666988 ) ;
#18102=EDGE_LOOP ( 'NONE', ( #49197, #81196 ) ) ;
#18103=VERTEX_POINT ( 'NONE', #58921 ) ;
#18104=CARTESIAN_POINT ( 'NONE',  ( 4.799999999999935874, 2.500000000000000000, 3.983716857408420964 ) ) ;
#18105=CARTESIAN_POINT ( 'NONE',  ( 0.6499999999999566125, 2.500000000000000000, -6.248780366869526759 ) ) ;
#18106=CARTESIAN_POINT ( 'NONE',  ( -8.550000000000013145, 2.500000000000000000, 2.511473670974873507 ) ) ;
#18107=CARTESIAN_POINT ( 'NONE',  ( -6.050000000000018474, 2.500000000000000000, 2.611473670974873151 ) ) ;
#18108=CARTESIAN_POINT ( 'NONE',  ( 14.34999999999989306, 12.50000000000000000, -2.511473670974877948 ) ) ;
#18109=CONICAL_SURFACE ( 'NONE', #28591, 0.1000000000000002554, 0.003490658503988666988 ) ;
#18110=DIRECTION ( 'NONE',  ( 0.000000000000000000, 0.000000000000000000, 1.000000000000000000 ) ) ;
#18111=CIRCLE ( 'NONE', #53626, 0.1000000000000002554 ) ;
#18112=CARTESIAN_POINT ( 'NONE',  ( -7.100000000000017408, 12.50000000000000000, -3.702399969078687292 ) ) ;
#18113=DIRECTION ( 'NONE',  ( 0.000000000000000000, 0.000000000000000000, -1.000000000000000000 ) ) ;
#18115=CARTESIAN_POINT ( 'NONE',  ( -11.04999999999999893, 2.500000000000000000, 6.148780366869520009 ) ) ;
#18116=AXIS2_PLACEMENT_3D ( 'NONE', #81247, #10546, #30871 ) ;
#18117=AXIS2_PLACEMENT_3D ( 'NONE', #35415, #115893, #96243 ) ;
#18118=CONICAL_SURFACE ( 'NONE', #36925, 0.09999999999999999167, 0.003490658503988666988 ) ;
#18119=ORIENTED_EDGE ( 'NONE', *, *, #34591, .F. ) ;
#18120=DIRECTION ( 'NONE',  ( 0.000000000000000000, 0.000000000000000000, 1.000000000000000000 ) ) ;
#18121=CARTESIAN_POINT ( 'NONE',  ( -1.250000000000036193, 12.50000000000000000, 5.867463478539781896 ) ) ;
#18122=DIRECTION ( 'NONE',  ( 0.000000000000000000, 0.000000000000000000, -1.000000000000000000 ) ) ;
#18123=CARTESIAN_POINT ( 'NONE',  ( 4.149999999999938183, 2.500000000000000000, 5.802370205355744659 ) ) ;
#18124=LINE ( 'NONE', #118911, #1979 ) ;
#18125=ORIENTED_EDGE ( 'NONE', *, *, #48102, .T. ) ;
#18126=CARTESIAN_POINT ( 'NONE',  ( -10.20000000000000462, 2.500000000000000000, 0.3464101615137735735 ) ) ;
#18127=EDGE_CURVE ( 'NONE', #17235, #101758, #40172, .T. ) ;
#18128=EDGE_CURVE ( 'NONE', #14173, #63919, #109090, .T. ) ;
#18129=CARTESIAN_POINT ( 'NONE',  ( 13.29999999999989946, 2.500000000000000000, -2.385244779468109755E-15 ) ) ;
#18130=CARTESIAN_POINT ( 'NONE',  ( -3.749999999999991118, 12.50000000000000000, 2.165063509461097713 ) ) ;
#18131=ORIENTED_EDGE ( 'NONE', *, *, #129246, .T. ) ;
#18132=AXIS2_PLACEMENT_3D ( 'NONE', #105148, #84872, #115609 ) ;
#18133=AXIS2_PLACEMENT_3D ( 'NONE', #77307, #107411, #45931 ) ;
#18134=ORIENTED_EDGE ( 'NONE', *, *, #110149, .F. ) ;
#18135=CIRCLE ( 'NONE', #87090, 0.06509327318403745899 ) ;
#18136=ADVANCED_FACE ( 'NONE', ( #110592 ), #40604, .T. ) ;
#18137=DIRECTION ( 'NONE',  ( 0.000000000000000000, 1.000000000000000000, 0.000000000000000000 ) ) ;
#18138=CIRCLE ( 'NONE', #95424, 0.09999999999999982514 ) ;
#18139=ORIENTED_EDGE ( 'NONE', *, *, #123478, .T. ) ;
#18140=ORIENTED_EDGE ( 'NONE', *, *, #78684, .T. ) ;
#18141=VERTEX_POINT ( 'NONE', #60234 ) ;
#18142=PLANE ( 'NONE',  #76161 ) ;
#18143=CIRCLE ( 'NONE', #93374, 0.09999999999999982514 ) ;
#18144=DIRECTION ( 'NONE',  ( -4.274815082592931898E-19, -0.9999939076577903929, -0.003490651415223739937 ) ) ;
#18145=CARTESIAN_POINT ( 'NONE',  ( -6.517459502904499961E-15, 2.500000000000000000, 4.230127018922196669 ) ) ;
#18146=AXIS2_PLACEMENT_3D ( 'NONE', #58780, #60718, #39802 ) ;
#18147=DIRECTION ( 'NONE',  ( -0.000000000000000000, -1.000000000000000000, -0.000000000000000000 ) ) ;
#18148=VERTEX_POINT ( 'NONE', #78580 ) ;
#18149=FACE_OUTER_BOUND ( 'NONE', #5077, .T. ) ;
#18150=ORIENTED_EDGE ( 'NONE', *, *, #35367, .F. ) ;
#18151=CARTESIAN_POINT ( 'NONE',  ( -4.999999999999986677, 2.500000000000000000, 4.330127018922196314 ) ) ;
#18152=DIRECTION ( 'NONE',  ( -0.000000000000000000, -1.000000000000000000, -0.000000000000000000 ) ) ;
#18153=CARTESIAN_POINT ( 'NONE',  ( 20.80581321129286820, 0.6997403544445329748, 4.161084241360442526 ) ) ;
#18155=AXIS2_PLACEMENT_3D ( 'NONE', #75861, #73942, #105337 ) ;
#18156=LINE ( 'NONE', #88835, #78898 ) ;
#18158=EDGE_LOOP ( 'NONE', ( #43913, #31774 ) ) ;
#18159=AXIS2_PLACEMENT_3D ( 'NONE', #29218, #118221, #39052 ) ;
#18160=CONICAL_SURFACE ( 'NONE', #34920, 0.09999999999999982514, 0.003490658503988666988 ) ;
#18161=ORIENTED_EDGE ( 'NONE', *, *, #14099, .T. ) ;
#18162=VERTEX_POINT ( 'NONE', #70035 ) ;
#18163=ORIENTED_EDGE ( 'NONE', *, *, #1237, .F. ) ;
#18164=VERTEX_POINT ( 'NONE', #79217 ) ;
#18165=CARTESIAN_POINT ( 'NONE',  ( 1.449999999999951328, 12.50000000000000000, -1.753560074763288679 ) ) ;
#18166=DIRECTION ( 'NONE',  ( -4.274815082592931898E-19, -0.9999939076577903929, -0.003490651415223739937 ) ) ;
#18167=DIRECTION ( 'NONE',  ( -0.000000000000000000, -1.000000000000000000, -0.000000000000000000 ) ) ;
#18168=FACE_BOUND ( 'NONE', #26367, .T. ) ;
#18169=CARTESIAN_POINT ( 'NONE',  ( -7.900000000000011013, 12.50000000000000000, 4.330127018922196314 ) ) ;
#18171=CARTESIAN_POINT ( 'NONE',  ( 12.49999999999990230, 2.500000000000000000, -0.5928203230275541635 ) ) ;
#18172=DIRECTION ( 'NONE',  ( -0.000000000000000000, -1.000000000000000000, -0.000000000000000000 ) ) ;
#18173=EDGE_CURVE ( 'NONE', #73698, #2826, #89029, .T. ) ;
#18174=LINE ( 'NONE', #88181, #8669 ) ;
#18175=CARTESIAN_POINT ( 'NONE',  ( -11.69999999999999574, 2.500000000000000000, 4.330127018922196314 ) ) ;
#18176=AXIS2_PLACEMENT_3D ( 'NONE', #103236, #44968, #52842 ) ;
#18177=CARTESIAN_POINT ( 'NONE',  ( -12.29999999999999361, 12.50000000000000000, 3.918623584224382839 ) ) ;
#18178=DIRECTION ( 'NONE',  ( 0.000000000000000000, 0.000000000000000000, 1.000000000000000000 ) ) ;
#18179=VERTEX_POINT ( 'NONE', #31407 ) ;
#18180=ORIENTED_EDGE ( 'NONE', *, *, #13810, .F. ) ;
#18181=VERTEX_POINT ( 'NONE', #71306 ) ;
#18182=ORIENTED_EDGE ( 'NONE', *, *, #83808, .T. ) ;
#18184=CARTESIAN_POINT ( 'NONE',  ( -12.29999999999999538, 2.500000000000000000, -0.3464101615137741841 ) ) ;
#18185=ADVANCED_FACE ( 'NONE', ( #30772 ), #50621, .T. ) ;
#18186=FACE_BOUND ( 'NONE', #54726, .T. ) ;
#18187=DIRECTION ( 'NONE',  ( 0.000000000000000000, 0.000000000000000000, 1.000000000000000000 ) ) ;
#18188=AXIS2_PLACEMENT_3D ( 'NONE', #81034, #90843, #9709 ) ;
#18189=VECTOR ( 'NONE', #103953, 1000.000000000000000 ) ;
#18190=ORIENTED_EDGE ( 'NONE', *, *, #31431, .F. ) ;
#18191=CARTESIAN_POINT ( 'NONE',  ( 12.49999999999990408, 2.500000000000000000, -3.637306695894650055 ) ) ;
#18192=EDGE_CURVE ( 'NONE', #49438, #39786, #123762, .T. ) ;
#18193=DIRECTION ( 'NONE',  ( 0.000000000000000000, 0.000000000000000000, 1.000000000000000000 ) ) ;
#18194=DIRECTION ( 'NONE',  ( -0.000000000000000000, 1.000000000000000000, -0.000000000000000000 ) ) ;
#18195=ORIENTED_EDGE ( 'NONE', *, *, #28914, .T. ) ;
#18197=CARTESIAN_POINT ( 'NONE',  ( -8.749999999999975131, 2.500000000000000000, -2.165063509461101710 ) ) ;
#18198=CONICAL_SURFACE ( 'NONE', #47457, 0.09999999999999982514, 0.003490658503988666988 ) ;
#18199=VERTEX_POINT ( 'NONE', #119770 ) ;
#18200=VERTEX_POINT ( 'NONE', #99500 ) ;
#18201=FACE_OUTER_BOUND ( 'NONE', #37724, .T. ) ;
#18202=LINE ( 'NONE', #99364, #87312 ) ;
#18203=CONICAL_SURFACE ( 'NONE', #108095, 0.09999999999999982514, 0.003490658503988666988 ) ;
#18204=AXIS2_PLACEMENT_3D ( 'NONE', #37828, #77112, #56165 ) ;
#18205=CIRCLE ( 'NONE', #70454, 0.06509327318403745899 ) ;
#18206=FACE_OUTER_BOUND ( 'NONE', #55944, .T. ) ;
#18207=CARTESIAN_POINT ( 'NONE',  ( -3.950000000000025491, 2.500000000000000000, 6.148780366869520897 ) ) ;
#18208=ORIENTED_EDGE ( 'NONE', *, *, #100951, .T. ) ;
#18209=CARTESIAN_POINT ( 'NONE',  ( -5.850000000000021849, 12.50000000000000000, -7.188010851410854052 ) ) ;
#18210=ORIENTED_EDGE ( 'NONE', *, *, #77205, .T. ) ;
#18211=ORIENTED_EDGE ( 'NONE', *, *, #106865, .T. ) ;
#18212=PLANE ( 'NONE',  #82831 ) ;
#18213=ORIENTED_EDGE ( 'NONE', *, *, #16417, .T. ) ;
#18214=FACE_OUTER_BOUND ( 'NONE', #65451, .T. ) ;
#18215=FACE_BOUND ( 'NONE', #1387, .T. ) ;
#18216=EDGE_CURVE ( 'NONE', #107817, #73591, #67314, .T. ) ;
#18217=VERTEX_POINT ( 'NONE', #90287 ) ;
#18218=DIRECTION ( 'NONE',  ( 0.000000000000000000, 0.000000000000000000, 1.000000000000000000 ) ) ;
#18219=EDGE_LOOP ( 'NONE', ( #82439, #99029, #12563, #69681 ) ) ;
#18221=DIRECTION ( 'NONE',  ( 0.000000000000000000, 0.000000000000000000, -1.000000000000000000 ) ) ;
#18222=CARTESIAN_POINT ( 'NONE',  ( -4.600000000000028955, 12.50000000000000000, -4.330127018922201643 ) ) ;
#18223=DIRECTION ( 'NONE',  ( 0.000000000000000000, 0.000000000000000000, -1.000000000000000000 ) ) ;
#18224=EDGE_CURVE ( 'NONE', #55568, #29710, #10882, .T. ) ;
#18225=EDGE_CURVE ( 'NONE', #63575, #17352, #71549, .T. ) ;
#18226=CARTESIAN_POINT ( 'NONE',  ( -3.750000000000027978, 2.500000000000000000, 7.188010851410848723 ) ) ;
#18227=VECTOR ( 'NONE', #672, 1000.000000000000000 ) ;
#18228=EDGE_CURVE ( 'NONE', #100677, #17818, #119561, .T. ) ;
#18229=ORIENTED_EDGE ( 'NONE', *, *, #68139, .T. ) ;
#18230=CONICAL_SURFACE ( 'NONE', #95515, 0.09999999999999982514, 0.003490658503988666988 ) ;
#18231=VERTEX_POINT ( 'NONE', #1282 ) ;
#18232=ORIENTED_EDGE ( 'NONE', *, *, #97775, .T. ) ;
#18233=CARTESIAN_POINT ( 'NONE',  ( -3.350000000000028955, 12.50000000000000000, 5.802370205355744659 ) ) ;
#18234=CIRCLE ( 'NONE', #105979, 1.000000000000000888 ) ;
#18236=EDGE_CURVE ( 'NONE', #99110, #16061, #109302, .T. ) ;
#18237=CARTESIAN_POINT ( 'NONE',  ( -5.800000000000018474, 2.500000000000000000, -2.276824562219559311E-15 ) ) ;
#18238=VERTEX_POINT ( 'NONE', #41234 ) ;
#18239=VERTEX_POINT ( 'NONE', #79840 ) ;
#18240=ADVANCED_FACE ( 'NONE', ( #50385 ), #15081, .T. ) ;
#18241=ORIENTED_EDGE ( 'NONE', *, *, #99401, .F. ) ;
#18242=EDGE_CURVE ( 'NONE', #118223, #2269, #88255, .T. ) ;
#18243=CARTESIAN_POINT ( 'NONE',  ( -12.04999999999999716, 2.500000000000000000, -6.395190528383298378 ) ) ;
#18244=CIRCLE ( 'NONE', #49565, 0.1000000000000002554 ) ;
#18245=DIRECTION ( 'NONE',  ( 0.000000000000000000, 0.000000000000000000, 1.000000000000000000 ) ) ;
#18246=CIRCLE ( 'NONE', #129097, 0.06509327318403745899 ) ;
#18247=ADVANCED_FACE ( 'NONE', ( #22878 ), #124292, .T. ) ;
#18248=DIRECTION ( 'NONE',  ( -0.000000000000000000, -1.000000000000000000, -0.000000000000000000 ) ) ;
#18249=FACE_OUTER_BOUND ( 'NONE', #25815, .T. ) ;
#18250=FACE_OUTER_BOUND ( 'NONE', #71532, .T. ) ;
#18251=DIRECTION ( 'NONE',  ( 0.000000000000000000, -0.9999939076577903929, 0.003490651415223739937 ) ) ;
#18252=DIRECTION ( 'NONE',  ( 0.000000000000000000, 0.000000000000000000, 1.000000000000000000 ) ) ;
#18253=AXIS2_PLACEMENT_3D ( 'NONE', #72512, #519, #73146 ) ;
#18254=EDGE_CURVE ( 'NONE', #113689, #117544, #63431, .T. ) ;
#18255=CARTESIAN_POINT ( 'NONE',  ( -11.05000000000000071, 2.500000000000000000, 2.411473670974873862 ) ) ;
#18256=EDGE_CURVE ( 'NONE', #10201, #90888, #41873, .T. ) ;
#18257=VERTEX_POINT ( 'NONE', #102071 ) ;
#18258=ORIENTED_EDGE ( 'NONE', *, *, #63108, .T. ) ;
#18259=CARTESIAN_POINT ( 'NONE',  ( 11.44999999999990870, 12.50000000000000000, 6.841600689897072485 ) ) ;
#18260=AXIS2_PLACEMENT_3D ( 'NONE', #48052, #79448, #87941 ) ;
#18261=AXIS2_PLACEMENT_3D ( 'NONE', #26910, #107398, #127680 ) ;
#18262=DIRECTION ( 'NONE',  ( -0.000000000000000000, 1.000000000000000000, -0.000000000000000000 ) ) ;
#18263=ORIENTED_EDGE ( 'NONE', *, *, #66578, .T. ) ;
#18264=ORIENTED_EDGE ( 'NONE', *, *, #44062, .F. ) ;
#18265=DIRECTION ( 'NONE',  ( 0.000000000000000000, 0.000000000000000000, 1.000000000000000000 ) ) ;
#18266=LINE ( 'NONE', #8433, #3006 ) ;
#18267=CARTESIAN_POINT ( 'NONE',  ( 2.500000000000002220, 2.500000000000000000, -8.999999999999998224 ) ) ;
#18268=CARTESIAN_POINT ( 'NONE',  ( 2.949999999999946887, 2.500000000000000000, -2.165063509461101710 ) ) ;
#18269=CARTESIAN_POINT ( 'NONE',  ( 9.999999999999948486, 2.500000000000000000, 4.230127018922196669 ) ) ;
#18270=CARTESIAN_POINT ( 'NONE',  ( 1.849999999999950573, 2.500000000000000000, -1.918653347947326004 ) ) ;
#18271=LINE ( 'NONE', #88277, #94952 ) ;
#18272=ORIENTED_EDGE ( 'NONE', *, *, #8320, .F. ) ;
#18273=DIRECTION ( 'NONE',  ( -4.274815082592931898E-19, -0.9999939076577903929, -0.003490651415223739937 ) ) ;
#18274=CARTESIAN_POINT ( 'NONE',  ( -8.350000000000013856, 12.50000000000000000, 2.165063509461097713 ) ) ;
#18276=EDGE_LOOP ( 'NONE', ( #17802, #46649 ) ) ;
#18277=ORIENTED_EDGE ( 'NONE', *, *, #127724, .F. ) ;
#18278=ORIENTED_EDGE ( 'NONE', *, *, #62154, .T. ) ;
#18279=ORIENTED_EDGE ( 'NONE', *, *, #27682, .T. ) ;
#18280=DIRECTION ( 'NONE',  ( 0.000000000000000000, 0.000000000000000000, 1.000000000000000000 ) ) ;
#18281=CARTESIAN_POINT ( 'NONE',  ( -4.999999999999986677, 12.50000000000000000, 4.395220292106234439 ) ) ;
#18282=ORIENTED_EDGE ( 'NONE', *, *, #71655, .T. ) ;
#18283=AXIS2_PLACEMENT_3D ( 'NONE', #110808, #101650, #12600 ) ;
#18284=CARTESIAN_POINT ( 'NONE',  ( 4.999999999999973355, 2.500000000000000000, -4.330127018922201643 ) ) ;
#18285=ADVANCED_FACE ( 'NONE', ( #71978 ), #101426, .T. ) ;
#18286=CONICAL_SURFACE ( 'NONE', #26611, 0.1000000000000002554, 0.003490658503988666988 ) ;
#18287=CARTESIAN_POINT ( 'NONE',  ( -0.8000000000000315747, 2.500000000000000000, -0.1000000000000000056 ) ) ;
#18289=CARTESIAN_POINT ( 'NONE',  ( -11.44999999999999929, 12.50000000000000000, -6.213873640053560798 ) ) ;
#18291=ORIENTED_EDGE ( 'NONE', *, *, #23658, .T. ) ;
#18292=CARTESIAN_POINT ( 'NONE',  ( 4.399999999999937295, 2.500000000000000000, 3.883716857408421319 ) ) ;
#18293=AXIS2_PLACEMENT_3D ( 'NONE', #74507, #94143, #81736 ) ;
#18294=CIRCLE ( 'NONE', #47558, 0.06509327318403745899 ) ;
#18295=LINE ( 'NONE', #48405, #127325 ) ;
#18296=VERTEX_POINT ( 'NONE', #33974 ) ;
#18297=AXIS2_PLACEMENT_3D ( 'NONE', #35486, #5994, #114668 ) ;
#18298=ORIENTED_EDGE ( 'NONE', *, *, #92546, .T. ) ;
#18299=ORIENTED_EDGE ( 'NONE', *, *, #111934, .F. ) ;
#18300=DIRECTION ( 'NONE',  ( -0.000000000000000000, -1.000000000000000000, -0.000000000000000000 ) ) ;
#18301=VECTOR ( 'NONE', #63861, 1000.000000000000000 ) ;
#18302=DIRECTION ( 'NONE',  ( -0.000000000000000000, -1.000000000000000000, -0.000000000000000000 ) ) ;
#18303=VECTOR ( 'NONE', #30306, 1000.000000000000000 ) ;
#18304=ORIENTED_EDGE ( 'NONE', *, *, #3179, .T. ) ;
#18305=FACE_OUTER_BOUND ( 'NONE', #116311, .T. ) ;
#18306=DIRECTION ( 'NONE',  ( 0.000000000000000000, 1.000000000000000000, 0.000000000000000000 ) ) ;
#18307=LINE ( 'NONE', #49732, #73449 ) ;
#18308=FACE_OUTER_BOUND ( 'NONE', #94748, .T. ) ;
#18309=ORIENTED_EDGE ( 'NONE', *, *, #39436, .T. ) ;
#18310=CONICAL_SURFACE ( 'NONE', #58046, 0.1000000000000002554, 0.003490658503988666988 ) ;
#18311=CARTESIAN_POINT ( 'NONE',  ( -5.850000000000018296, 2.500000000000000000, 7.088010851410848190 ) ) ;
#18312=VECTOR ( 'NONE', #39523, 1000.000000000000000 ) ;
#18313=ORIENTED_EDGE ( 'NONE', *, *, #81965, .T. ) ;
#18314=ORIENTED_EDGE ( 'NONE', *, *, #48811, .F. ) ;
#18315=DIRECTION ( 'NONE',  ( 0.000000000000000000, 0.000000000000000000, -1.000000000000000000 ) ) ;
#18316=CARTESIAN_POINT ( 'NONE',  ( 12.69999999999990337, 12.50000000000000000, 3.918623584224382839 ) ) ;
#18317=FACE_BOUND ( 'NONE', #109209, .T. ) ;
#18318=AXIS2_PLACEMENT_3D ( 'NONE', #114192, #44155, #121574 ) ;
#18320=CARTESIAN_POINT ( 'NONE',  ( -9.150000000000005684, 2.500000000000000000, 7.288010851410849256 ) ) ;
#18321=CONICAL_SURFACE ( 'NONE', #72628, 0.1000000000000002554, 0.003490658503988666988 ) ;
#18322=DIRECTION ( 'NONE',  ( -0.000000000000000000, -1.000000000000000000, -0.000000000000000000 ) ) ;
#18323=ADVANCED_FACE ( 'NONE', ( #53615 ), #109194, .T. ) ;
#18324=CONICAL_SURFACE ( 'NONE', #64302, 0.1000000000000002554, 0.003490658503988666988 ) ;
#18325=EDGE_LOOP ( 'NONE', ( #97508, #90310, #95408, #74436 ) ) ;
#18326=CARTESIAN_POINT ( 'NONE',  ( 13.34999999999989662, 12.50000000000000000, -2.165063509461101710 ) ) ;
#18327=DIRECTION ( 'NONE',  ( -0.000000000000000000, -1.000000000000000000, -0.000000000000000000 ) ) ;
#18328=AXIS2_PLACEMENT_3D ( 'NONE', #107571, #17218, #86631 ) ;
#18329=CARTESIAN_POINT ( 'NONE',  ( 3.549999999999942091, 2.500000000000000000, 2.611473670974873151 ) ) ;
#18330=VECTOR ( 'NONE', #41589, 1000.000000000000000 ) ;
#18331=CARTESIAN_POINT ( 'NONE',  ( 12.49999999999990585, 2.500000000000000000, 3.637306695894644726 ) ) ;
#18332=ORIENTED_EDGE ( 'NONE', *, *, #75975, .F. ) ;
#18333=EDGE_CURVE ( 'NONE', #113637, #4728, #44453, .T. ) ;
#18335=CIRCLE ( 'NONE', #62272, 0.1000000000000002554 ) ;
#18336=CARTESIAN_POINT ( 'NONE',  ( 5.849999999999933031, 2.500000000000000000, -1.472243186433550122 ) ) ;
#18337=VERTEX_POINT ( 'NONE', #12388 ) ;
#18338=ORIENTED_EDGE ( 'NONE', *, *, #36366, .T. ) ;
#18339=EDGE_CURVE ( 'NONE', #109623, #97511, #71644, .T. ) ;
#18340=DIRECTION ( 'NONE',  ( 0.000000000000000000, 1.000000000000000000, 0.000000000000000000 ) ) ;
#18341=AXIS2_PLACEMENT_3D ( 'NONE', #77636, #46916, #86821 ) ;
#18342=DIRECTION ( 'NONE',  ( -0.000000000000000000, -1.000000000000000000, -0.000000000000000000 ) ) ;
#18343=EDGE_CURVE ( 'NONE', #91438, #1733, #121811, .T. ) ;
#18344=FACE_BOUND ( 'NONE', #116469, .T. ) ;
#18345=DIRECTION ( 'NONE',  ( -0.000000000000000000, 1.000000000000000000, -0.000000000000000000 ) ) ;
#18346=VECTOR ( 'NONE', #112773, 1000.000000000000000 ) ;
#18347=CIRCLE ( 'NONE', #30896, 0.06509327318403743123 ) ;
#18348=ORIENTED_EDGE ( 'NONE', *, *, #106890, .F. ) ;
#18349=DIRECTION ( 'NONE',  ( 0.000000000000000000, -0.9999939076577903929, 0.003490651415223739937 ) ) ;
#18350=ADVANCED_FACE ( 'NONE', ( #22234 ), #84147, .T. ) ;
#18351=VERTEX_POINT ( 'NONE', #122364 ) ;
#18352=EDGE_LOOP ( 'NONE', ( #2743, #71828, #43374, #21440 ) ) ;
#18353=DIRECTION ( 'NONE',  ( -0.000000000000000000, -1.000000000000000000, -0.000000000000000000 ) ) ;
#18354=ADVANCED_FACE ( 'NONE', ( #72614 ), #83724, .T. ) ;
#18356=EDGE_LOOP ( 'NONE', ( #43369, #15357 ) ) ;
#18357=DIRECTION ( 'NONE',  ( 0.000000000000000000, 1.000000000000000000, 0.000000000000000000 ) ) ;
#18358=DIRECTION ( 'NONE',  ( -0.000000000000000000, 1.000000000000000000, -0.000000000000000000 ) ) ;
#18359=DIRECTION ( 'NONE',  ( 0.000000000000000000, 1.000000000000000000, 0.000000000000000000 ) ) ;
#18361=EDGE_LOOP ( 'NONE', ( #30333, #105550, #57019, #45940 ) ) ;
#18363=CARTESIAN_POINT ( 'NONE',  ( 0.3999999999999555023, 12.50000000000000000, 4.265033745738159077 ) ) ;
#18364=CARTESIAN_POINT ( 'NONE',  ( -2.950000000000033484, 2.500000000000000000, -6.395190528383301931 ) ) ;
#18365=FACE_OUTER_BOUND ( 'NONE', #2741, .T. ) ;
#18366=EDGE_LOOP ( 'NONE', ( #28978, #91898 ) ) ;
#18367=CONICAL_SURFACE ( 'NONE', #7991, 0.1000000000000002554, 0.003490658503988666988 ) ;
#18368=FACE_OUTER_BOUND ( 'NONE', #109675, .T. ) ;
#18369=ORIENTED_EDGE ( 'NONE', *, *, #65350, .T. ) ;
#18370=CARTESIAN_POINT ( 'NONE',  ( -13.29999999999999005, 12.50000000000000000, 1.843143693225357538E-15 ) ) ;
#18371=EDGE_LOOP ( 'NONE', ( #24524, #56209, #102658, #96120 ) ) ;
#18372=CARTESIAN_POINT ( 'NONE',  ( 7.499999999999961808, 2.500000000000000000, 4.330127018922196314 ) ) ;
#18373=CARTESIAN_POINT ( 'NONE',  ( 87.50000000000002842, -4.424430252271037922, 6.079088403633667426 ) ) ;
#18374=VECTOR ( 'NONE', #95052, 1000.000000000000000 ) ;
#18375=EDGE_CURVE ( 'NONE', #31757, #37517, #50714, .T. ) ;
#18376=FACE_OUTER_BOUND ( 'NONE', #11796, .T. ) ;
#18377=AXIS2_PLACEMENT_3D ( 'NONE', #111339, #2044, #82564 ) ;
#18378=CARTESIAN_POINT ( 'NONE',  ( -4.150000000000025224, 12.50000000000000000, -1.472243186433550122 ) ) ;
#18379=ORIENTED_EDGE ( 'NONE', *, *, #35690, .F. ) ;
#18380=CARTESIAN_POINT ( 'NONE',  ( -14.14999999999998792, 12.50000000000000000, -1.472243186433547901 ) ) ;
#18381=DIRECTION ( 'NONE',  ( 0.000000000000000000, 0.000000000000000000, 1.000000000000000000 ) ) ;
#18384=DIRECTION ( 'NONE',  ( -4.274815082592931898E-19, -0.9999939076577903929, -0.003490651415223739937 ) ) ;
#18385=EDGE_CURVE ( 'NONE', #95311, #103899, #2668, .T. ) ;
#18386=LINE ( 'NONE', #66195, #3439 ) ;
#18387=AXIS2_PLACEMENT_3D ( 'NONE', #6168, #5525, #46112 ) ;
#18388=EDGE_CURVE ( 'NONE', #82453, #118813, #73249, .T. ) ;
#18389=ORIENTED_EDGE ( 'NONE', *, *, #34101, .T. ) ;
#18390=AXIS2_PLACEMENT_3D ( 'NONE', #111121, #71884, #119671 ) ;
#18391=AXIS2_PLACEMENT_3D ( 'NONE', #120404, #32038, #90934 ) ;
#18392=ORIENTED_EDGE ( 'NONE', *, *, #128930, .F. ) ;
#18393=DIRECTION ( 'NONE',  ( -0.000000000000000000, 1.000000000000000000, -0.000000000000000000 ) ) ;
#18394=ORIENTED_EDGE ( 'NONE', *, *, #122754, .T. ) ;
#18395=CARTESIAN_POINT ( 'NONE',  ( 0.8499999999999553468, 2.500000000000000000, 2.265063509461097357 ) ) ;
#18396=EDGE_CURVE ( 'NONE', #33188, #51687, #67405, .T. ) ;
#18397=ORIENTED_EDGE ( 'NONE', *, *, #20447, .F. ) ;
#18398=ORIENTED_EDGE ( 'NONE', *, *, #59197, .F. ) ;
#18399=ADVANCED_FACE ( 'NONE', ( #92910 ), #113167, .T. ) ;
#18400=ORIENTED_EDGE ( 'NONE', *, *, #61378, .F. ) ;
#18401=EDGE_CURVE ( 'NONE', #26037, #37993, #73683, .T. ) ;
#18402=DIRECTION ( 'NONE',  ( -4.274815082592931898E-19, -0.9999939076577903929, -0.003490651415223739937 ) ) ;
#18403=EDGE_CURVE ( 'NONE', #28723, #103868, #86269, .T. ) ;
#18404=CIRCLE ( 'NONE', #45518, 0.06509327318403741736 ) ;
#18405=LINE ( 'NONE', #100194, #90353 ) ;
#18406=FACE_OUTER_BOUND ( 'NONE', #4447, .T. ) ;
#18407=ADVANCED_FACE ( 'NONE', ( #24798 ), #111328, .T. ) ;
#18408=CARTESIAN_POINT ( 'NONE',  ( 2.499999999999948930, 2.500000000000000000, -0.5928203230275541635 ) ) ;
#18409=FACE_OUTER_BOUND ( 'NONE', #55341, .T. ) ;
#18410=DIRECTION ( 'NONE',  ( 0.000000000000000000, 0.000000000000000000, 1.000000000000000000 ) ) ;
#18411=AXIS2_PLACEMENT_3D ( 'NONE', #97167, #37616, #120036 ) ;
#18412=DIRECTION ( 'NONE',  ( 0.000000000000000000, 0.000000000000000000, 1.000000000000000000 ) ) ;
#18413=CARTESIAN_POINT ( 'NONE',  ( 0.8499999999999553468, 2.500000000000000000, -2.065063509461102065 ) ) ;
#18414=EDGE_CURVE ( 'NONE', #101138, #123793, #119664, .T. ) ;
#18415=ORIENTED_EDGE ( 'NONE', *, *, #43569, .F. ) ;
#18416=AXIS2_PLACEMENT_3D ( 'NONE', #88177, #28002, #8989 ) ;
#18417=EDGE_CURVE ( 'NONE', #64400, #55444, #124929, .T. ) ;
#18418=VERTEX_POINT ( 'NONE', #7064 ) ;
#18419=ORIENTED_EDGE ( 'NONE', *, *, #32499, .F. ) ;
#18420=DIRECTION ( 'NONE',  ( -0.000000000000000000, -1.000000000000000000, -0.000000000000000000 ) ) ;
#18421=VERTEX_POINT ( 'NONE', #35904 ) ;
#18422=EDGE_LOOP ( 'NONE', ( #105222, #21950 ) ) ;
#18423=CARTESIAN_POINT ( 'NONE',  ( 11.69999999999990514, 2.500000000000000000, 0.09999999999999772959 ) ) ;
#18426=FACE_OUTER_BOUND ( 'NONE', #65842, .T. ) ;
#18427=DIRECTION ( 'NONE',  ( -0.000000000000000000, 1.000000000000000000, -0.000000000000000000 ) ) ;
#18428=AXIS2_PLACEMENT_3D ( 'NONE', #53899, #124574, #64354 ) ;
#18429=DIRECTION ( 'NONE',  ( -4.274815082592931898E-19, -0.9999939076577903929, -0.003490651415223739937 ) ) ;
#18430=FACE_OUTER_BOUND ( 'NONE', #100945, .T. ) ;
#18431=DIRECTION ( 'NONE',  ( -0.000000000000000000, 1.000000000000000000, -0.000000000000000000 ) ) ;
#18432=EDGE_LOOP ( 'NONE', ( #101870, #113375 ) ) ;
#18433=AXIS2_PLACEMENT_3D ( 'NONE', #101628, #12574, #121898 ) ;
#18434=CARTESIAN_POINT ( 'NONE',  ( 6.049999999999934097, 12.50000000000000000, -6.213873640053564351 ) ) ;
#18435=EDGE_LOOP ( 'NONE', ( #7434, #100166, #57505, #13627 ) ) ;
#18436=DIRECTION ( 'NONE',  ( 0.000000000000000000, 0.000000000000000000, -1.000000000000000000 ) ) ;
#18437=ORIENTED_EDGE ( 'NONE', *, *, #97032, .T. ) ;
#18438=DIRECTION ( 'NONE',  ( 0.000000000000000000, 0.000000000000000000, 1.000000000000000000 ) ) ;
#18439=ORIENTED_EDGE ( 'NONE', *, *, #123322, .T. ) ;
#18440=CONICAL_SURFACE ( 'NONE', #39400, 0.1000000000000002554, 0.003490658503988666988 ) ;
#18441=VERTEX_POINT ( 'NONE', #14935 ) ;
#18442=CARTESIAN_POINT ( 'NONE',  ( 9.799999999999913669, 12.50000000000000000, -3.983716857408426293 ) ) ;
#18443=DIRECTION ( 'NONE',  ( 0.000000000000000000, 1.000000000000000000, 0.000000000000000000 ) ) ;
#18444=CIRCLE ( 'NONE', #22667, 0.06509327318403745899 ) ;
#18445=DIRECTION ( 'NONE',  ( 0.000000000000000000, 0.000000000000000000, -1.000000000000000000 ) ) ;
#18446=ADVANCED_FACE ( 'NONE', ( #26728 ), #40262, .T. ) ;
#18447=CARTESIAN_POINT ( 'NONE',  ( 7.899999999999921307, 2.500000000000000000, -2.385244779468109755E-15 ) ) ;
#18448=CARTESIAN_POINT ( 'NONE',  ( -8.150000000000012790, 2.500000000000000000, -1.918653347947326004 ) ) ;
#18449=ORIENTED_EDGE ( 'NONE', *, *, #13194, .T. ) ;
#18451=FACE_OUTER_BOUND ( 'NONE', #120222, .T. ) ;
#18452=CARTESIAN_POINT ( 'NONE',  ( 5.399999999999934630, 2.500000000000000000, -0.5928203230275542746 ) ) ;
#18453=DIRECTION ( 'NONE',  ( -4.274815082592931898E-19, -0.9999939076577903929, -0.003490651415223739937 ) ) ;
#18454=CARTESIAN_POINT ( 'NONE',  ( 3.349999999999941025, 2.500000000000000000, 7.188010851410848723 ) ) ;
#18455=DIRECTION ( 'NONE',  ( 0.000000000000000000, 0.000000000000000000, 1.000000000000000000 ) ) ;
#18456=EDGE_CURVE ( 'NONE', #100810, #19127, #96105, .T. ) ;
#18457=ORIENTED_EDGE ( 'NONE', *, *, #93178, .T. ) ;
#18458=ORIENTED_EDGE ( 'NONE', *, *, #48377, .T. ) ;
#18459=CIRCLE ( 'NONE', #60339, 0.09999999999999982514 ) ;
#18460=FACE_OUTER_BOUND ( 'NONE', #33792, .T. ) ;
#18461=ORIENTED_EDGE ( 'NONE', *, *, #26133, .F. ) ;
#18462=DIRECTION ( 'NONE',  ( 0.000000000000000000, 0.000000000000000000, 1.000000000000000000 ) ) ;
#18463=DIRECTION ( 'NONE',  ( -0.000000000000000000, 1.000000000000000000, -0.000000000000000000 ) ) ;
#18464=CIRCLE ( 'NONE', #102378, 0.06509327318403745899 ) ;
#18465=AXIS2_PLACEMENT_3D ( 'NONE', #39850, #28726, #50294 ) ;
#18466=EDGE_LOOP ( 'NONE', ( #73540, #39509, #62442, #18721 ) ) ;
#18468=DIRECTION ( 'NONE',  ( 0.000000000000000000, 0.000000000000000000, 1.000000000000000000 ) ) ;
#18469=DIRECTION ( 'NONE',  ( -0.000000000000000000, -1.000000000000000000, -0.000000000000000000 ) ) ;
#18470=CARTESIAN_POINT ( 'NONE',  ( -9.600000000000006750, 12.50000000000000000, 4.957854068765711553 ) ) ;
#18471=ORIENTED_EDGE ( 'NONE', *, *, #121181, .F. ) ;
#18472=CIRCLE ( 'NONE', #91628, 0.09999999999999999167 ) ;
#18473=CONICAL_SURFACE ( 'NONE', #14261, 0.1000000000000002554, 0.003490658503988666988 ) ;
#18475=VERTEX_POINT ( 'NONE', #25417 ) ;
#18476=PLANE ( 'NONE',  #109117 ) ;
#18477=DIRECTION ( 'NONE',  ( 0.000000000000000000, 0.000000000000000000, 1.000000000000000000 ) ) ;
#18478=AXIS2_PLACEMENT_3D ( 'NONE', #43791, #104611, #103984 ) ;
#18479=DIRECTION ( 'NONE',  ( 0.000000000000000000, 0.000000000000000000, 1.000000000000000000 ) ) ;
#18480=CIRCLE ( 'NONE', #108366, 0.06509327318403745899 ) ;
#18481=VERTEX_POINT ( 'NONE', #5144 ) ;
#18482=CARTESIAN_POINT ( 'NONE',  ( -1.650000000000034328, 2.500000000000000000, -2.857883832488653741 ) ) ;
#18483=VERTEX_POINT ( 'NONE', #66639 ) ;
#18484=CARTESIAN_POINT ( 'NONE',  ( -12.69999999999999218, 12.50000000000000000, -4.741630453620012453 ) ) ;
#18485=CARTESIAN_POINT ( 'NONE',  ( -5.650000000000023448, 2.500000000000000000, -6.941600689897078347 ) ) ;
#18486=DIRECTION ( 'NONE',  ( 0.000000000000000000, 0.000000000000000000, -1.000000000000000000 ) ) ;
#18487=ORIENTED_EDGE ( 'NONE', *, *, #95960, .T. ) ;
#18488=AXIS2_PLACEMENT_3D ( 'NONE', #61535, #91620, #41898 ) ;
#18490=CARTESIAN_POINT ( 'NONE',  ( 4.999999999999935163, 12.50000000000000000, 0.6928203230275494784 ) ) ;
#18491=CARTESIAN_POINT ( 'NONE',  ( 8.749999999999920064, 12.50000000000000000, -2.857883832488653741 ) ) ;
#18492=AXIS2_PLACEMENT_3D ( 'NONE', #4739, #84620, #35529 ) ;
#18493=ORIENTED_EDGE ( 'NONE', *, *, #86362, .F. ) ;
#18494=EDGE_CURVE ( 'NONE', #125159, #14617, #117585, .T. ) ;
#18495=CARTESIAN_POINT ( 'NONE',  ( -8.350000000000013856, 12.50000000000000000, -6.560283801567334372 ) ) ;
#18496=EDGE_CURVE ( 'NONE', #64737, #89101, #6772, .T. ) ;
#18497=ORIENTED_EDGE ( 'NONE', *, *, #36520, .F. ) ;
#18498=DIRECTION ( 'NONE',  ( 0.000000000000000000, 0.000000000000000000, 1.000000000000000000 ) ) ;
#18499=AXIS2_PLACEMENT_3D ( 'NONE', #88957, #19567, #38589 ) ;
#18500=VERTEX_POINT ( 'NONE', #7712 ) ;
#18501=DIRECTION ( 'NONE',  ( 0.000000000000000000, 1.000000000000000000, 0.000000000000000000 ) ) ;
#18502=DIRECTION ( 'NONE',  ( -0.000000000000000000, 1.000000000000000000, -0.000000000000000000 ) ) ;
#18503=EDGE_CURVE ( 'NONE', #2195, #72665, #27724, .T. ) ;
#18504=EDGE_LOOP ( 'NONE', ( #118652, #11125, #92586, #39286 ) ) ;
#18505=ORIENTED_EDGE ( 'NONE', *, *, #22569, .T. ) ;
#18506=EDGE_CURVE ( 'NONE', #32289, #64667, #79958, .T. ) ;
#18507=CARTESIAN_POINT ( 'NONE',  ( 8.749999999999953815, 12.50000000000000000, 6.495190528383297135 ) ) ;
#18508=CARTESIAN_POINT ( 'NONE',  ( -12.89999999999999147, 2.500000000000000000, -0.09999999999999815981 ) ) ;
#18509=AXIS2_PLACEMENT_3D ( 'NONE', #52701, #92631, #124019 ) ;
#18510=VERTEX_POINT ( 'NONE', #16236 ) ;
#18511=LINE ( 'NONE', #79380, #126240 ) ;
#18513=AXIS2_PLACEMENT_3D ( 'NONE', #103482, #123126, #23627 ) ;
#18514=DIRECTION ( 'NONE',  ( 0.000000000000000000, 0.000000000000000000, 1.000000000000000000 ) ) ;
#18516=LINE ( 'NONE', #86606, #103190 ) ;
#18517=DIRECTION ( 'NONE',  ( -0.000000000000000000, -1.000000000000000000, -0.000000000000000000 ) ) ;
#18518=DIRECTION ( 'NONE',  ( 0.000000000000000000, 1.000000000000000000, 0.000000000000000000 ) ) ;
#18519=CIRCLE ( 'NONE', #100007, 0.06509327318403745899 ) ;
#18520=ORIENTED_EDGE ( 'NONE', *, *, #99106, .T. ) ;
#18521=ORIENTED_EDGE ( 'NONE', *, *, #82137, .T. ) ;
#18522=VERTEX_POINT ( 'NONE', #56172 ) ;
#18523=EDGE_LOOP ( 'NONE', ( #45384, #50290 ) ) ;
#18524=DIRECTION ( 'NONE',  ( -4.274815082592931898E-19, -0.9999939076577903929, -0.003490651415223739937 ) ) ;
#18526=FACE_OUTER_BOUND ( 'NONE', #72709, .T. ) ;
#18527=AXIS2_PLACEMENT_3D ( 'NONE', #120277, #49613, #20137 ) ;
#18528=ORIENTED_EDGE ( 'NONE', *, *, #128148, .F. ) ;
#18529=FACE_BOUND ( 'NONE', #81500, .T. ) ;
#18530=EDGE_LOOP ( 'NONE', ( #24570, #41127, #88867, #29475 ) ) ;
#18531=DIRECTION ( 'NONE',  ( -4.274815082592931898E-19, -0.9999939076577903929, -0.003490651415223739937 ) ) ;
#18532=DIRECTION ( 'NONE',  ( -0.000000000000000000, 1.000000000000000000, -0.000000000000000000 ) ) ;
#18533=CARTESIAN_POINT ( 'NONE',  ( -5.650000000000019895, 2.500000000000000000, 2.611473670974873151 ) ) ;
#18534=AXIS2_PLACEMENT_3D ( 'NONE', #113503, #63776, #103700 ) ;
#18535=CONICAL_SURFACE ( 'NONE', #68704, 0.1000000000000002554, 0.003490658503988666988 ) ;
#18536=DIRECTION ( 'NONE',  ( 0.000000000000000000, 0.000000000000000000, 1.000000000000000000 ) ) ;
#18537=CARTESIAN_POINT ( 'NONE',  ( 16.32066102237038052, -2.500000000000000000, -4.877377760480627877 ) ) ;
#18538=CARTESIAN_POINT ( 'NONE',  ( -6.650000000000019007, 12.50000000000000000, -1.537336459617587581 ) ) ;
#18539=LINE ( 'NONE', #119309, #22722 ) ;
#18540=LINE ( 'NONE', #58492, #9569 ) ;
#18541=CARTESIAN_POINT ( 'NONE',  ( 2.949999999999943334, 12.50000000000000000, 6.430097255199259010 ) ) ;
#18542=DIRECTION ( 'NONE',  ( 0.000000000000000000, 0.000000000000000000, -1.000000000000000000 ) ) ;
#18543=ORIENTED_EDGE ( 'NONE', *, *, #127627, .F. ) ;
#18544=ORIENTED_EDGE ( 'NONE', *, *, #123486, .F. ) ;
#18545=EDGE_LOOP ( 'NONE', ( #39049, #36035, #61146, #4149 ) ) ;
#18547=DIRECTION ( 'NONE',  ( 0.000000000000000000, 0.000000000000000000, 1.000000000000000000 ) ) ;
#18548=EDGE_CURVE ( 'NONE', #128192, #58954, #36151, .T. ) ;
#18549=AXIS2_PLACEMENT_3D ( 'NONE', #104638, #112553, #75192 ) ;
#18550=DIRECTION ( 'NONE',  ( -0.000000000000000000, 1.000000000000000000, -0.000000000000000000 ) ) ;
#18551=ADVANCED_FACE ( 'NONE', ( #47027 ), #128087, .T. ) ;
#18552=ORIENTED_EDGE ( 'NONE', *, *, #128642, .F. ) ;
#18553=ORIENTED_EDGE ( 'NONE', *, *, #93943, .T. ) ;
#18554=ORIENTED_EDGE ( 'NONE', *, *, #42349, .F. ) ;
#18555=EDGE_CURVE ( 'NONE', #3435, #13662, #100877, .T. ) ;
#18557=AXIS2_PLACEMENT_3D ( 'NONE', #113117, #90908, #52280 ) ;
#18558=CONICAL_SURFACE ( 'NONE', #85450, 0.09999999999999982514, 0.003490658503988666988 ) ;
#18559=PLANE ( 'NONE',  #80184 ) ;
#18561=AXIS2_PLACEMENT_3D ( 'NONE', #46926, #113726, #105180 ) ;
#18562=PLANE ( 'NONE',  #73084 ) ;
#18563=ADVANCED_FACE ( 'NONE', ( #87567 ), #127511, .T. ) ;
#18564=CARTESIAN_POINT ( 'NONE',  ( -1.050000000000038236, 12.50000000000000000, -1.883746621131363597 ) ) ;
#18565=CARTESIAN_POINT ( 'NONE',  ( -8.749999999999975131, 2.500000000000000000, -2.165063509461101710 ) ) ;
#18566=CARTESIAN_POINT ( 'NONE',  ( 7.299999999999927880, 2.500000000000000000, -4.676537180435977881 ) ) ;
#18567=ORIENTED_EDGE ( 'NONE', *, *, #46424, .T. ) ;
#18568=VECTOR ( 'NONE', #116449, 1000.000000000000000 ) ;
#18569=DIRECTION ( 'NONE',  ( -0.000000000000000000, 1.000000000000000000, -0.000000000000000000 ) ) ;
#18570=ADVANCED_FACE ( 'NONE', ( #77741 ), #28020, .T. ) ;
#18571=ORIENTED_EDGE ( 'NONE', *, *, #91259, .F. ) ;
#18572=AXIS2_PLACEMENT_3D ( 'NONE', #104544, #74446, #6957 ) ;
#18573=EDGE_CURVE ( 'NONE', #120803, #38135, #109805, .T. ) ;
#18574=EDGE_LOOP ( 'NONE', ( #75497, #6215, #88448, #25602 ) ) ;
#18575=VERTEX_POINT ( 'NONE', #79066 ) ;
#18576=CARTESIAN_POINT ( 'NONE',  ( 11.04999999999990656, 2.500000000000000000, -6.048780366869526581 ) ) ;
#18577=ORIENTED_EDGE ( 'NONE', *, *, #79558, .F. ) ;
#18578=EDGE_LOOP ( 'NONE', ( #32570, #122849, #77306, #110469 ) ) ;
#18579=EDGE_CURVE ( 'NONE', #10886, #29292, #36053, .T. ) ;
#18580=AXIS2_PLACEMENT_3D ( 'NONE', #9490, #57952, #107021 ) ;
#18581=DIRECTION ( 'NONE',  ( -0.000000000000000000, -1.000000000000000000, -0.000000000000000000 ) ) ;
#18582=AXIS2_PLACEMENT_3D ( 'NONE', #69977, #39250, #118417 ) ;
#18583=LINE ( 'NONE', #77495, #7790 ) ;
#18584=FACE_OUTER_BOUND ( 'NONE', #74217, .T. ) ;
#18585=CARTESIAN_POINT ( 'NONE',  ( -7.500000000000015099, 12.50000000000000000, -5.022947341949754119 ) ) ;
#18586=DIRECTION ( 'NONE',  ( -0.000000000000000000, -1.000000000000000000, -0.000000000000000000 ) ) ;
#18587=VERTEX_POINT ( 'NONE', #118972 ) ;
#18588=CARTESIAN_POINT ( 'NONE',  ( 10.19999999999991047, 2.500000000000000000, 4.776537180435972196 ) ) ;
#18589=CIRCLE ( 'NONE', #91745, 0.1000000000000002554 ) ;
#18590=VERTEX_POINT ( 'NONE', #40437 ) ;
#18591=CARTESIAN_POINT ( 'NONE',  ( 11.24999999999994316, 2.500000000000000000, 2.165063509461097713 ) ) ;
#18592=EDGE_LOOP ( 'NONE', ( #18571, #54827, #20337, #94269 ) ) ;
#18593=CARTESIAN_POINT ( 'NONE',  ( -3.750000000000027534, 2.500000000000000000, -1.472243186433550122 ) ) ;
#18594=DIRECTION ( 'NONE',  ( 0.000000000000000000, -0.000000000000000000, 1.000000000000000000 ) ) ;
#18595=VECTOR ( 'NONE', #108752, 1000.000000000000000 ) ;
#18596=ORIENTED_EDGE ( 'NONE', *, *, #55304, .T. ) ;
#18597=CARTESIAN_POINT ( 'NONE',  ( 10.64999999999990976, 2.500000000000000000, -6.148780366869526226 ) ) ;
#18598=DIRECTION ( 'NONE',  ( -0.000000000000000000, 1.000000000000000000, -0.000000000000000000 ) ) ;
#18599=EDGE_LOOP ( 'NONE', ( #71382, #127309, #21671, #99524 ) ) ;
#18600=AXIS2_PLACEMENT_3D ( 'NONE', #23255, #52728, #103119 ) ;
#18601=DIRECTION ( 'NONE',  ( 0.000000000000000000, 0.000000000000000000, 1.000000000000000000 ) ) ;
#18602=VERTEX_POINT ( 'NONE', #117653 ) ;
#18603=EDGE_LOOP ( 'NONE', ( #115761, #6895, #34353, #38959 ) ) ;
#18604=DIRECTION ( 'NONE',  ( -0.000000000000000000, -1.000000000000000000, -0.000000000000000000 ) ) ;
#18605=DIRECTION ( 'NONE',  ( 1.000000000000000000, 0.000000000000000000, 0.000000000000000000 ) ) ;
#18607=DIRECTION ( 'NONE',  ( 0.000000000000000000, 0.000000000000000000, 1.000000000000000000 ) ) ;
#18608=AXIS2_PLACEMENT_3D ( 'NONE', #33709, #113558, #91985 ) ;
#18609=AXIS2_PLACEMENT_3D ( 'NONE', #48426, #7194, #118448 ) ;
#18610=CARTESIAN_POINT ( 'NONE',  ( -11.25000000000000178, 2.500000000000000000, -5.702370205355745902 ) ) ;
#18611=ADVANCED_FACE ( 'NONE', ( #107861 ), #105071, .T. ) ;
#18612=CARTESIAN_POINT ( 'NONE',  ( 0.6499999999999543920, 2.500000000000000000, 6.148780366869520897 ) ) ;
#18613=AXIS2_PLACEMENT_3D ( 'NONE', #1640, #112263, #42897 ) ;
#18614=ORIENTED_EDGE ( 'NONE', *, *, #85736, .F. ) ;
#18615=CARTESIAN_POINT ( 'NONE',  ( 2.499999999999945377, 2.500000000000000000, 5.122947341949749323 ) ) ;
#18616=FACE_OUTER_BOUND ( 'NONE', #37833, .T. ) ;
#18617=EDGE_LOOP ( 'NONE', ( #45672, #41954 ) ) ;
#18618=AXIS2_PLACEMENT_3D ( 'NONE', #121043, #91588, #42504 ) ;
#18619=CIRCLE ( 'NONE', #27035, 0.06509327318403745899 ) ;
#18620=CARTESIAN_POINT ( 'NONE',  ( -1.650000000000034328, 12.50000000000000000, -2.857883832488653741 ) ) ;
#18621=DIRECTION ( 'NONE',  ( 0.000000000000000000, 0.000000000000000000, 1.000000000000000000 ) ) ;
#18622=DIRECTION ( 'NONE',  ( 0.000000000000000000, 0.000000000000000000, -1.000000000000000000 ) ) ;
#18623=DIRECTION ( 'NONE',  ( 0.000000000000000000, 0.000000000000000000, 1.000000000000000000 ) ) ;
#18624=DIRECTION ( 'NONE',  ( -0.000000000000000000, 1.000000000000000000, -0.000000000000000000 ) ) ;
#18626=AXIS2_PLACEMENT_3D ( 'NONE', #112466, #120984, #120351 ) ;
#18627=CIRCLE ( 'NONE', #81336, 0.09999999999999982514 ) ;
#18628=DIRECTION ( 'NONE',  ( -0.000000000000000000, 1.000000000000000000, -0.000000000000000000 ) ) ;
#18629=ORIENTED_EDGE ( 'NONE', *, *, #105223, .F. ) ;
#18630=DIRECTION ( 'NONE',  ( 0.000000000000000000, -0.000000000000000000, 1.000000000000000000 ) ) ;
#18631=EDGE_LOOP ( 'NONE', ( #75650, #39003 ) ) ;
#18632=EDGE_LOOP ( 'NONE', ( #59240, #78890, #16554, #124288 ) ) ;
#18633=LINE ( 'NONE', #88672, #111462 ) ;
#18634=VECTOR ( 'NONE', #124625, 1000.000000000000000 ) ;
#18635=ORIENTED_EDGE ( 'NONE', *, *, #96176, .F. ) ;
#18636=CARTESIAN_POINT ( 'NONE',  ( 9.799999999999913669, 12.50000000000000000, 4.676537180435972552 ) ) ;
#18637=FACE_OUTER_BOUND ( 'NONE', #28058, .T. ) ;
#18638=EDGE_LOOP ( 'NONE', ( #126585, #120510, #32192, #24815 ) ) ;
#18639=ADVANCED_FACE ( 'NONE', ( #8361 ), #13035, .T. ) ;
#18640=CARTESIAN_POINT ( 'NONE',  ( 1.649999999999951505, 2.500000000000000000, -1.472243186433550122 ) ) ;
#18641=AXIS2_PLACEMENT_3D ( 'NONE', #28105, #37921, #56888 ) ;
#18642=CARTESIAN_POINT ( 'NONE',  ( 6.649999999999927525, 2.500000000000000000, 2.265063509461097357 ) ) ;
#18643=ORIENTED_EDGE ( 'NONE', *, *, #94948, .F. ) ;
#18644=DIRECTION ( 'NONE',  ( -4.274815082592931898E-19, -0.9999939076577903929, -0.003490651415223739937 ) ) ;
#18645=EDGE_CURVE ( 'NONE', #120001, #97971, #88194, .T. ) ;
#18646=CARTESIAN_POINT ( 'NONE',  ( 10.19999999999991580, 12.50000000000000000, -0.3464101615137783474 ) ) ;
#18647=EDGE_CURVE ( 'NONE', #115023, #127206, #105181, .T. ) ;
#18648=AXIS2_PLACEMENT_3D ( 'NONE', #56584, #57249, #116155 ) ;
#18649=ORIENTED_EDGE ( 'NONE', *, *, #12144, .T. ) ;
#18650=CIRCLE ( 'NONE', #31289, 0.09999999999999999167 ) ;
#18651=AXIS2_PLACEMENT_3D ( 'NONE', #127082, #46560, #37414 ) ;
#18652=ORIENTED_EDGE ( 'NONE', *, *, #75545, .F. ) ;
#18653=ORIENTED_EDGE ( 'NONE', *, *, #40994, .T. ) ;
#18654=DIRECTION ( 'NONE',  ( 0.000000000000000000, 1.000000000000000000, 0.000000000000000000 ) ) ;
#18655=CARTESIAN_POINT ( 'NONE',  ( -5.450000000000019718, 12.50000000000000000, 2.165063509461097713 ) ) ;
#18656=EDGE_CURVE ( 'NONE', #98821, #43976, #99989, .T. ) ;
#18657=EDGE_CURVE ( 'NONE', #121861, #1292, #128155, .T. ) ;
#18658=LINE ( 'NONE', #116849, #100694 ) ;
#18659=ADVANCED_FACE ( 'NONE', ( #78433 ), #67508, .T. ) ;
#18660=FACE_BOUND ( 'NONE', #119961, .T. ) ;
#18661=EDGE_LOOP ( 'NONE', ( #42686, #18232 ) ) ;
#18662=ADVANCED_FACE ( 'NONE', ( #119610 ), #98928, .T. ) ;
#18663=ADVANCED_FACE ( 'NONE', ( #29960 ), #49610, .T. ) ;
#18664=CIRCLE ( 'NONE', #39626, 0.09999999999999999167 ) ;
#18665=DIRECTION ( 'NONE',  ( 0.000000000000000000, 0.000000000000000000, -1.000000000000000000 ) ) ;
#18666=LINE ( 'NONE', #89346, #68977 ) ;
#18667=ORIENTED_EDGE ( 'NONE', *, *, #68463, .T. ) ;
#18669=FACE_OUTER_BOUND ( 'NONE', #9388, .T. ) ;
#18670=DIRECTION ( 'NONE',  ( -0.000000000000000000, -1.000000000000000000, -0.000000000000000000 ) ) ;
#18671=CARTESIAN_POINT ( 'NONE',  ( -7.500000000000015099, 12.50000000000000000, -0.6277270498435166823 ) ) ;
#18672=DIRECTION ( 'NONE',  ( 0.000000000000000000, 0.000000000000000000, 1.000000000000000000 ) ) ;
#18673=EDGE_CURVE ( 'NONE', #23087, #107893, #13132, .T. ) ;
#18674=DIRECTION ( 'NONE',  ( -4.274815082592931898E-19, -0.9999939076577903929, -0.003490651415223739937 ) ) ;
#18675=DIRECTION ( 'NONE',  ( 0.000000000000000000, 1.000000000000000000, 0.000000000000000000 ) ) ;
#18676=VERTEX_POINT ( 'NONE', #70511 ) ;
#18677=ORIENTED_EDGE ( 'NONE', *, *, #20763, .T. ) ;
#18678=ORIENTED_EDGE ( 'NONE', *, *, #121124, .T. ) ;
#18679=ORIENTED_EDGE ( 'NONE', *, *, #74890, .F. ) ;
#18680=VERTEX_POINT ( 'NONE', #79689 ) ;
#18681=AXIS2_PLACEMENT_3D ( 'NONE', #86210, #80286, #79628 ) ;
#18682=CARTESIAN_POINT ( 'NONE',  ( 9.999999999999912959, 2.500000000000000000, 3.537306695894645081 ) ) ;
#18683=DIRECTION ( 'NONE',  ( 0.000000000000000000, 1.000000000000000000, 0.000000000000000000 ) ) ;
#18684=ORIENTED_EDGE ( 'NONE', *, *, #634, .F. ) ;
#18685=FACE_BOUND ( 'NONE', #82515, .T. ) ;
#18686=DIRECTION ( 'NONE',  ( 0.000000000000000000, 0.000000000000000000, -1.000000000000000000 ) ) ;
#18687=DIRECTION ( 'NONE',  ( 0.000000000000000000, 1.000000000000000000, 0.000000000000000000 ) ) ;
#18688=DIRECTION ( 'NONE',  ( 0.000000000000000000, -0.000000000000000000, 1.000000000000000000 ) ) ;
#18689=CARTESIAN_POINT ( 'NONE',  ( -1.450000000000036371, 12.50000000000000000, 2.511473670974873507 ) ) ;
#18690=CARTESIAN_POINT ( 'NONE',  ( -2.950000000000030376, 2.500000000000000000, 6.495190528383297135 ) ) ;
#18691=ORIENTED_EDGE ( 'NONE', *, *, #1378, .F. ) ;
#18692=AXIS2_PLACEMENT_3D ( 'NONE', #36141, #46592, #27582 ) ;
#18693=EDGE_LOOP ( 'NONE', ( #84986, #79542, #2009, #96102 ) ) ;
#18694=ORIENTED_EDGE ( 'NONE', *, *, #89057, .T. ) ;
#18695=ORIENTED_EDGE ( 'NONE', *, *, #72, .F. ) ;
#18696=CARTESIAN_POINT ( 'NONE',  ( -5.000000000000023093, 12.50000000000000000, 5.022947341949748790 ) ) ;
#18697=CARTESIAN_POINT ( 'NONE',  ( 8.920123399827135202, 2.500000000000000444, 8.410822907074514632 ) ) ;
#18698=DIRECTION ( 'NONE',  ( 0.000000000000000000, 1.000000000000000000, 0.000000000000000000 ) ) ;
#18699=EDGE_CURVE ( 'NONE', #32827, #27222, #48762, .T. ) ;
#18700=AXIS2_PLACEMENT_3D ( 'NONE', #19182, #9396, #126592 ) ;
#18701=ORIENTED_EDGE ( 'NONE', *, *, #19892, .F. ) ;
#18702=CARTESIAN_POINT ( 'NONE',  ( -12.69999999999999218, 2.500000000000000000, 4.676537180435972552 ) ) ;
#18703=EDGE_CURVE ( 'NONE', #79119, #4868, #9005, .T. ) ;
#18704=FACE_OUTER_BOUND ( 'NONE', #12966, .T. ) ;
#18705=ADVANCED_FACE ( 'NONE', ( #467 ), #60708, .F. ) ;
#18706=VECTOR ( 'NONE', #27958, 1000.000000000000000 ) ;
#18707=LINE ( 'NONE', #107077, #60354 ) ;
#18708=CIRCLE ( 'NONE', #35446, 0.06509327318403745899 ) ;
#18710=FACE_OUTER_BOUND ( 'NONE', #35915, .T. ) ;
#18711=DIRECTION ( 'NONE',  ( 0.000000000000000000, 0.000000000000000000, 1.000000000000000000 ) ) ;
#18712=CIRCLE ( 'NONE', #121123, 0.06509327318403745899 ) ;
#18713=DIRECTION ( 'NONE',  ( 0.000000000000000000, 0.000000000000000000, -1.000000000000000000 ) ) ;
#18714=ADVANCED_FACE ( 'NONE', ( #83576 ), #34092, .T. ) ;
#18715=VERTEX_POINT ( 'NONE', #31254 ) ;
#18716=CARTESIAN_POINT ( 'NONE',  ( 1.249999999999952038, 2.500000000000000000, -1.472243186433550122 ) ) ;
#18717=EDGE_CURVE ( 'NONE', #94678, #26454, #42357, .T. ) ;
#18718=AXIS2_PLACEMENT_3D ( 'NONE', #69137, #10847, #61926 ) ;
#18719=AXIS2_PLACEMENT_3D ( 'NONE', #106377, #35083, #76280 ) ;
#18720=EDGE_CURVE ( 'NONE', #93687, #62761, #52870, .T. ) ;
#18721=ORIENTED_EDGE ( 'NONE', *, *, #86837, .F. ) ;
#18722=EDGE_CURVE ( 'NONE', #102277, #78527, #82208, .T. ) ;
#18723=VERTEX_POINT ( 'NONE', #111060 ) ;
#18724=DIRECTION ( 'NONE',  ( 0.000000000000000000, 0.000000000000000000, 1.000000000000000000 ) ) ;
#18725=CARTESIAN_POINT ( 'NONE',  ( 1.249999999999952038, 12.50000000000000000, -1.472243186433550122 ) ) ;
#18726=DIRECTION ( 'NONE',  ( 0.000000000000000000, 1.000000000000000000, 0.000000000000000000 ) ) ;
#18727=ORIENTED_EDGE ( 'NONE', *, *, #59483, .F. ) ;
#18728=ADVANCED_FACE ( 'NONE', ( #92079 ), #82928, .T. ) ;
#18729=ORIENTED_EDGE ( 'NONE', *, *, #31419, .T. ) ;
#18730=CARTESIAN_POINT ( 'NONE',  ( -7.100000000000014744, 2.500000000000000000, 4.430127018922196847 ) ) ;
#18731=DIRECTION ( 'NONE',  ( 0.000000000000000000, -0.000000000000000000, 1.000000000000000000 ) ) ;
#18732=CARTESIAN_POINT ( 'NONE',  ( 0.1999999999999571565, 2.500000000000000000, 3.983716857408420076 ) ) ;
#18733=CONICAL_SURFACE ( 'NONE', #102279, 0.1000000000000002554, 0.003490658503988666988 ) ;
#18734=EDGE_LOOP ( 'NONE', ( #114827, #10811 ) ) ;
#18735=ORIENTED_EDGE ( 'NONE', *, *, #106902, .T. ) ;
#18736=DIRECTION ( 'NONE',  ( -0.000000000000000000, -1.000000000000000000, -0.000000000000000000 ) ) ;
#18738=CARTESIAN_POINT ( 'NONE',  ( 6.249999999999928946, 2.500000000000000000, 2.857883832488649301 ) ) ;
#18739=ORIENTED_EDGE ( 'NONE', *, *, #80298, .F. ) ;
#18740=CARTESIAN_POINT ( 'NONE',  ( 5.649999999999932854, 2.500000000000000000, 1.818653347947321475 ) ) ;
#18743=EDGE_CURVE ( 'NONE', #12428, #99630, #29883, .T. ) ;
#18744=FACE_OUTER_BOUND ( 'NONE', #125110, .T. ) ;
#18745=AXIS2_PLACEMENT_3D ( 'NONE', #73500, #12008, #53239 ) ;
#18746=ORIENTED_EDGE ( 'NONE', *, *, #113890, .F. ) ;
#18747=AXIS2_PLACEMENT_3D ( 'NONE', #27134, #66401, #67029 ) ;
#18748=AXIS2_PLACEMENT_3D ( 'NONE', #20349, #119831, #108717 ) ;
#18749=ORIENTED_EDGE ( 'NONE', *, *, #118180, .F. ) ;
#18750=ORIENTED_EDGE ( 'NONE', *, *, #51539, .T. ) ;
#18751=CARTESIAN_POINT ( 'NONE',  ( -12.04999999999999538, 2.500000000000000000, 2.165063509461097713 ) ) ;
#18752=DIRECTION ( 'NONE',  ( 0.000000000000000000, 1.000000000000000000, 0.000000000000000000 ) ) ;
#18753=PLANE ( 'NONE',  #3025 ) ;
#18754=CARTESIAN_POINT ( 'NONE',  ( 8.149999999999920419, 2.500000000000000000, -2.611473670974877592 ) ) ;
#18755=CONICAL_SURFACE ( 'NONE', #50175, 0.1000000000000002554, 0.003490658503988666988 ) ;
#18756=DIRECTION ( 'NONE',  ( 0.000000000000000000, 0.000000000000000000, 1.000000000000000000 ) ) ;
#18757=CARTESIAN_POINT ( 'NONE',  ( 3.749999999999944045, 2.500000000000000000, -2.857883832488653741 ) ) ;
#18758=CONICAL_SURFACE ( 'NONE', #91922, 0.1000000000000000056, 0.003490658503988666988 ) ;
#18759=AXIS2_PLACEMENT_3D ( 'NONE', #103660, #15899, #13964 ) ;
#18760=DIRECTION ( 'NONE',  ( 0.000000000000000000, 0.000000000000000000, 1.000000000000000000 ) ) ;
#18761=EDGE_CURVE ( 'NONE', #123229, #35564, #71158, .T. ) ;
#18762=CARTESIAN_POINT ( 'NONE',  ( 12.09999999999990550, 12.50000000000000000, -3.637306695894650055 ) ) ;
#18763=FACE_OUTER_BOUND ( 'NONE', #122110, .T. ) ;
#18764=DIRECTION ( 'NONE',  ( -0.000000000000000000, -1.000000000000000000, -0.000000000000000000 ) ) ;
#18765=AXIS2_PLACEMENT_3D ( 'NONE', #26860, #34765, #46486 ) ;
#18766=ORIENTED_EDGE ( 'NONE', *, *, #106417, .F. ) ;
#18767=CIRCLE ( 'NONE', #68952, 0.06509327318403745899 ) ;
#18768=CARTESIAN_POINT ( 'NONE',  ( 11.64999999999990621, 12.50000000000000000, -2.165063509461101710 ) ) ;
#18770=DIRECTION ( 'NONE',  ( 0.000000000000000000, -0.000000000000000000, 1.000000000000000000 ) ) ;
#18771=DIRECTION ( 'NONE',  ( -0.000000000000000000, -1.000000000000000000, -0.000000000000000000 ) ) ;
#18772=DIRECTION ( 'NONE',  ( 0.000000000000000000, 1.000000000000000000, 0.000000000000000000 ) ) ;
#18773=DIRECTION ( 'NONE',  ( -0.000000000000000000, -1.000000000000000000, -0.000000000000000000 ) ) ;
#18774=VERTEX_POINT ( 'NONE', #33194 ) ;
#18775=DIRECTION ( 'NONE',  ( 0.000000000000000000, 0.000000000000000000, 1.000000000000000000 ) ) ;
#18776=LINE ( 'NONE', #56120, #65867 ) ;
#18777=CARTESIAN_POINT ( 'NONE',  ( -14.39999999999998614, 2.500000000000000000, 0.3464101615137758494 ) ) ;
#18778=ORIENTED_EDGE ( 'NONE', *, *, #77905, .T. ) ;
#18779=ORIENTED_EDGE ( 'NONE', *, *, #6397, .T. ) ;
#18781=ORIENTED_EDGE ( 'NONE', *, *, #3234, .F. ) ;
#18782=ORIENTED_EDGE ( 'NONE', *, *, #30336, .T. ) ;
#18783=ORIENTED_EDGE ( 'NONE', *, *, #14336, .F. ) ;
#18784=LINE ( 'NONE', #38456, #103359 ) ;
#18785=CIRCLE ( 'NONE', #91962, 0.1000000000000002554 ) ;
#18786=LINE ( 'NONE', #127468, #117744 ) ;
#18787=DIRECTION ( 'NONE',  ( 0.000000000000000000, -0.000000000000000000, 1.000000000000000000 ) ) ;
#18788=CARTESIAN_POINT ( 'NONE',  ( 16.87640210516320138, 2.500000000000000000, -4.436424697255190175 ) ) ;
#18789=VERTEX_POINT ( 'NONE', #14156 ) ;
#18790=EDGE_CURVE ( 'NONE', #123810, #56755, #52172, .T. ) ;
#18791=CIRCLE ( 'NONE', #91965, 0.06509327318403745899 ) ;
#18792=AXIS2_PLACEMENT_3D ( 'NONE', #47492, #56002, #97227 ) ;
#18793=PLANE ( 'NONE',  #33612 ) ;
#18794=ORIENTED_EDGE ( 'NONE', *, *, #61825, .T. ) ;
#18795=DIRECTION ( 'NONE',  ( 0.000000000000000000, 0.000000000000000000, 1.000000000000000000 ) ) ;
#18796=CARTESIAN_POINT ( 'NONE',  ( 19.40342015654457342, -2.551666867761286817, -4.359384978533091370 ) ) ;
#18797=DIRECTION ( 'NONE',  ( -0.000000000000000000, 1.000000000000000000, -0.000000000000000000 ) ) ;
#18798=CARTESIAN_POINT ( 'NONE',  ( -3.950000000000026379, 2.500000000000000000, -1.818653347947326138 ) ) ;
#18799=DIRECTION ( 'NONE',  ( 0.000000000000000000, 0.000000000000000000, 1.000000000000000000 ) ) ;
#18800=EDGE_LOOP ( 'NONE', ( #112911, #17433, #117356, #114410 ) ) ;
#18801=VECTOR ( 'NONE', #51948, 1000.000000000000000 ) ;
#18802=AXIS2_PLACEMENT_3D ( 'NONE', #85767, #34113, #4609 ) ;
#18803=ORIENTED_EDGE ( 'NONE', *, *, #115388, .T. ) ;
#18804=ORIENTED_EDGE ( 'NONE', *, *, #236, .T. ) ;
#18805=ORIENTED_EDGE ( 'NONE', *, *, #20304, .T. ) ;
#18806=EDGE_LOOP ( 'NONE', ( #117930, #95849 ) ) ;
#18807=DIRECTION ( 'NONE',  ( -0.000000000000000000, -1.000000000000000000, -0.000000000000000000 ) ) ;
#18808=CARTESIAN_POINT ( 'NONE',  ( -3.950000000000029932, 2.500000000000000000, -6.248780366869526759 ) ) ;
#18809=EDGE_CURVE ( 'NONE', #8036, #87854, #43654, .T. ) ;
#18810=EDGE_CURVE ( 'NONE', #48591, #91335, #92744, .T. ) ;
#18811=DIRECTION ( 'NONE',  ( 0.000000000000000000, 0.000000000000000000, 1.000000000000000000 ) ) ;
#18812=EDGE_CURVE ( 'NONE', #116552, #39180, #46601, .T. ) ;
#18813=FACE_BOUND ( 'NONE', #69035, .T. ) ;
#18814=ADVANCED_FACE ( 'NONE', ( #94022 ), #96758, .T. ) ;
#18815=CARTESIAN_POINT ( 'NONE',  ( 8.549999999999920774, 12.50000000000000000, 6.148780366869520897 ) ) ;
#18817=DIRECTION ( 'NONE',  ( 0.000000000000000000, -0.9999939076577903929, 0.003490651415223739937 ) ) ;
#18818=CARTESIAN_POINT ( 'NONE',  ( -1.250000000000035749, 2.500000000000000000, -7.288010851410854585 ) ) ;
#18819=ADVANCED_FACE ( 'NONE', ( #111731 ), #22082, .T. ) ;
#18821=CARTESIAN_POINT ( 'NONE',  ( -2.050000000000033129, 2.500000000000000000, 6.495190528383297135 ) ) ;
#18822=EDGE_CURVE ( 'NONE', #29211, #23253, #73099, .T. ) ;
#18823=DIRECTION ( 'NONE',  ( -0.000000000000000000, -1.000000000000000000, -0.000000000000000000 ) ) ;
#18824=EDGE_CURVE ( 'NONE', #127460, #109714, #90510, .T. ) ;
#18825=AXIS2_PLACEMENT_3D ( 'NONE', #73299, #113222, #53669 ) ;
#18826=ADVANCED_FACE ( 'NONE', ( #63274 ), #61284, .T. ) ;
#18827=CARTESIAN_POINT ( 'NONE',  ( 13.14999999999989733, 12.50000000000000000, -2.446380397790840266 ) ) ;
#18828=VERTEX_POINT ( 'NONE', #124121 ) ;
#18829=ORIENTED_EDGE ( 'NONE', *, *, #98337, .T. ) ;
#18830=VERTEX_POINT ( 'NONE', #76323 ) ;
#18831=ORIENTED_EDGE ( 'NONE', *, *, #128245, .T. ) ;
#18832=DIRECTION ( 'NONE',  ( -0.000000000000000000, -1.000000000000000000, -0.000000000000000000 ) ) ;
#18833=CARTESIAN_POINT ( 'NONE',  ( -10.84999999999999964, 2.500000000000000000, 5.702370205355745014 ) ) ;
#18834=FACE_BOUND ( 'NONE', #26503, .T. ) ;
#18835=AXIS2_PLACEMENT_3D ( 'NONE', #106533, #29280, #98633 ) ;
#18836=LINE ( 'NONE', #16869, #1702 ) ;
#18837=VERTEX_POINT ( 'NONE', #126715 ) ;
#18838=CARTESIAN_POINT ( 'NONE',  ( 10.64999999999990976, 2.500000000000000000, -6.148780366869526226 ) ) ;
#18839=FACE_OUTER_BOUND ( 'NONE', #1758, .T. ) ;
#18840=FACE_OUTER_BOUND ( 'NONE', #90497, .T. ) ;
#18841=DIRECTION ( 'NONE',  ( 0.000000000000000000, 0.000000000000000000, 1.000000000000000000 ) ) ;
#18842=CIRCLE ( 'NONE', #58575, 0.1000000000000002554 ) ;
#18843=VERTEX_POINT ( 'NONE', #46868 ) ;
#18844=FACE_OUTER_BOUND ( 'NONE', #115321, .T. ) ;
#18845=CIRCLE ( 'NONE', #20912, 0.09999999999999982514 ) ;
#18846=AXIS2_PLACEMENT_3D ( 'NONE', #104140, #94971, #123759 ) ;
#18847=VERTEX_POINT ( 'NONE', #114938 ) ;
#18848=ORIENTED_EDGE ( 'NONE', *, *, #30128, .F. ) ;
#18849=CARTESIAN_POINT ( 'NONE',  ( -4.800000000000026468, 2.500000000000000000, -4.676537180435978769 ) ) ;
#18851=ORIENTED_EDGE ( 'NONE', *, *, #13405, .F. ) ;
#18852=VECTOR ( 'NONE', #100738, 1000.000000000000000 ) ;
#18853=CARTESIAN_POINT ( 'NONE',  ( -1.050000000000037348, 12.50000000000000000, -6.776507416713040577 ) ) ;
#18854=DIRECTION ( 'NONE',  ( 0.000000000000000000, 1.000000000000000000, 0.000000000000000000 ) ) ;
#18855=EDGE_LOOP ( 'NONE', ( #24640, #37583, #55404, #61190 ) ) ;
#18856=PLANE ( 'NONE',  #95420 ) ;
#18857=AXIS2_PLACEMENT_3D ( 'NONE', #114601, #124436, #24945 ) ;
#18858=EDGE_LOOP ( 'NONE', ( #129272, #65600 ) ) ;
#18859=FACE_OUTER_BOUND ( 'NONE', #43707, .T. ) ;
#18860=ORIENTED_EDGE ( 'NONE', *, *, #28487, .T. ) ;
#18861=FACE_OUTER_BOUND ( 'NONE', #15979, .T. ) ;
#18862=FACE_BOUND ( 'NONE', #88647, .T. ) ;
#18863=ADVANCED_FACE ( 'NONE', ( #106418 ), #5623, .T. ) ;
#18864=ORIENTED_EDGE ( 'NONE', *, *, #7739, .F. ) ;
#18865=CARTESIAN_POINT ( 'NONE',  ( 4.149999999999941735, 12.50000000000000000, -5.867463478539787225 ) ) ;
#18866=ADVANCED_FACE ( 'NONE', ( #104483 ), #121918, .T. ) ;
#18867=ORIENTED_EDGE ( 'NONE', *, *, #121524, .F. ) ;
#18868=DIRECTION ( 'NONE',  ( 0.000000000000000000, 0.000000000000000000, 1.000000000000000000 ) ) ;
#18869=DIRECTION ( 'NONE',  ( -0.000000000000000000, 1.000000000000000000, -0.000000000000000000 ) ) ;
#18870=PLANE ( 'NONE',  #36238 ) ;
#18871=CARTESIAN_POINT ( 'NONE',  ( -3.350000000000028955, 12.50000000000000000, 7.122917578226811486 ) ) ;
#18872=CARTESIAN_POINT ( 'NONE',  ( 10.79999999999991012, 12.50000000000000000, 4.330127018922196314 ) ) ;
#18873=VERTEX_POINT ( 'NONE', #75032 ) ;
#18874=EDGE_CURVE ( 'NONE', #14289, #112256, #44933, .T. ) ;
#18875=VERTEX_POINT ( 'NONE', #56019 ) ;
#18876=ORIENTED_EDGE ( 'NONE', *, *, #3488, .F. ) ;
#18877=DIRECTION ( 'NONE',  ( 0.000000000000000000, 1.000000000000000000, 0.000000000000000000 ) ) ;
#18878=PLANE ( 'NONE',  #57794 ) ;
#18879=CONICAL_SURFACE ( 'NONE', #127555, 0.09999999999999999167, 0.003490658503988666988 ) ;
#18880=DIRECTION ( 'NONE',  ( -0.000000000000000000, 1.000000000000000000, -0.000000000000000000 ) ) ;
#18881=EDGE_LOOP ( 'NONE', ( #98647, #103753 ) ) ;
#18882=ORIENTED_EDGE ( 'NONE', *, *, #3192, .F. ) ;
#18883=VERTEX_POINT ( 'NONE', #25261 ) ;
#18884=DIRECTION ( 'NONE',  ( 0.000000000000000000, 0.000000000000000000, 1.000000000000000000 ) ) ;
#18887=CONICAL_SURFACE ( 'NONE', #121304, 0.1000000000000002554, 0.003490658503988666988 ) ;
#18888=DIRECTION ( 'NONE',  ( 0.000000000000000000, 0.000000000000000000, -1.000000000000000000 ) ) ;
#18889=CARTESIAN_POINT ( 'NONE',  ( -10.85000000000000142, 2.500000000000000000, -1.472243186433546125 ) ) ;
#18890=CARTESIAN_POINT ( 'NONE',  ( -6.250000000000017764, 2.500000000000000000, 2.857883832488649301 ) ) ;
#18891=DIRECTION ( 'NONE',  ( -0.000000000000000000, -1.000000000000000000, -0.000000000000000000 ) ) ;
#18892=CARTESIAN_POINT ( 'NONE',  ( 0.8499999999999553468, 12.50000000000000000, -2.099970236277064473 ) ) ;
#18893=DIRECTION ( 'NONE',  ( 0.000000000000000000, -0.9999939076577903929, 0.003490651415223739937 ) ) ;
#18895=ORIENTED_EDGE ( 'NONE', *, *, #45238, .F. ) ;
#18896=DIRECTION ( 'NONE',  ( 0.000000000000000000, 1.000000000000000000, 0.000000000000000000 ) ) ;
#18897=DIRECTION ( 'NONE',  ( -4.274815082592931898E-19, -0.9999939076577903929, -0.003490651415223739937 ) ) ;
#18898=ORIENTED_EDGE ( 'NONE', *, *, #55092, .T. ) ;
#18899=ORIENTED_EDGE ( 'NONE', *, *, #12512, .T. ) ;
#18901=FACE_OUTER_BOUND ( 'NONE', #121687, .T. ) ;
#18902=DIRECTION ( 'NONE',  ( 0.000000000000000000, 0.000000000000000000, -1.000000000000000000 ) ) ;
#18903=DIRECTION ( 'NONE',  ( 0.000000000000000000, 0.000000000000000000, 1.000000000000000000 ) ) ;
#18904=CARTESIAN_POINT ( 'NONE',  ( -1.450000000000035483, 12.50000000000000000, 1.753560074763284016 ) ) ;
#18905=EDGE_CURVE ( 'NONE', #32401, #72821, #92668, .T. ) ;
#18906=CARTESIAN_POINT ( 'NONE',  ( 14.54999999999989235, 12.50000000000000000, -2.099970236277064473 ) ) ;
#18907=CARTESIAN_POINT ( 'NONE',  ( 7.299999999999926104, 2.500000000000000000, -0.3464101615137782364 ) ) ;
#18909=AXIS2_PLACEMENT_3D ( 'NONE', #49855, #89758, #11832 ) ;
#18910=AXIS2_PLACEMENT_3D ( 'NONE', #61425, #120964, #60763 ) ;
#18911=ORIENTED_EDGE ( 'NONE', *, *, #126272, .F. ) ;
#18912=ORIENTED_EDGE ( 'NONE', *, *, #48422, .F. ) ;
#18913=EDGE_CURVE ( 'NONE', #18680, #121502, #116231, .T. ) ;
#18914=VERTEX_POINT ( 'NONE', #4981 ) ;
#18915=EDGE_CURVE ( 'NONE', #60519, #66379, #94658, .T. ) ;
#18916=ORIENTED_EDGE ( 'NONE', *, *, #20304, .F. ) ;
#18917=DIRECTION ( 'NONE',  ( 0.000000000000000000, 1.000000000000000000, 0.000000000000000000 ) ) ;
#18918=PLANE ( 'NONE',  #24839 ) ;
#18919=CIRCLE ( 'NONE', #117189, 0.06509327318403745899 ) ;
#18920=ORIENTED_EDGE ( 'NONE', *, *, #65683, .T. ) ;
#18921=CARTESIAN_POINT ( 'NONE',  ( -10.60000000000000142, 2.500000000000000000, -0.4464101615137782142 ) ) ;
#18922=FACE_OUTER_BOUND ( 'NONE', #105195, .T. ) ;
#18923=PLANE ( 'NONE',  #26366 ) ;
#18924=DIRECTION ( 'NONE',  ( 0.000000000000000000, 1.000000000000000000, 0.000000000000000000 ) ) ;
#18925=VERTEX_POINT ( 'NONE', #6903 ) ;
#18926=ADVANCED_FACE ( 'NONE', ( #84194 ), #57055, .T. ) ;
#18927=CARTESIAN_POINT ( 'NONE',  ( 12.09999999999990550, 2.500000000000000000, 5.022947341949748790 ) ) ;
#18928=CARTESIAN_POINT ( 'NONE',  ( 5.199999999999933564, 12.50000000000000000, 0.3464101615137735735 ) ) ;
#18929=CIRCLE ( 'NONE', #112948, 0.1000000000000002554 ) ;
#18930=ORIENTED_EDGE ( 'NONE', *, *, #22410, .F. ) ;
#18931=AXIS2_PLACEMENT_3D ( 'NONE', #66618, #123601, #46335 ) ;
#18932=ORIENTED_EDGE ( 'NONE', *, *, #80789, .F. ) ;
#18933=EDGE_LOOP ( 'NONE', ( #10267, #14208, #79583, #89567 ) ) ;
#18934=ORIENTED_EDGE ( 'NONE', *, *, #46428, .T. ) ;
#18935=PLANE ( 'NONE',  #44775 ) ;
#18936=CIRCLE ( 'NONE', #44086, 0.06509327318403745899 ) ;
#18937=DIRECTION ( 'NONE',  ( 0.000000000000000000, 0.000000000000000000, 1.000000000000000000 ) ) ;
#18938=EDGE_CURVE ( 'NONE', #7520, #7926, #115579, .T. ) ;
#18939=AXIS2_PLACEMENT_3D ( 'NONE', #110279, #967, #119440 ) ;
#18941=DIRECTION ( 'NONE',  ( 0.000000000000000000, 1.000000000000000000, 0.000000000000000000 ) ) ;
#18942=LINE ( 'NONE', #95590, #7778 ) ;
#18943=DIRECTION ( 'NONE',  ( -0.000000000000000000, 1.000000000000000000, -0.000000000000000000 ) ) ;
#18944=DIRECTION ( 'NONE',  ( 0.000000000000000000, 1.000000000000000000, 0.000000000000000000 ) ) ;
#18945=ADVANCED_FACE ( 'NONE', ( #64557 ), #75931, .T. ) ;
#18946=VERTEX_POINT ( 'NONE', #34478 ) ;
#18947=DIRECTION ( 'NONE',  ( 0.000000000000000000, -0.000000000000000000, 1.000000000000000000 ) ) ;
#18948=EDGE_LOOP ( 'NONE', ( #76792, #113315 ) ) ;
#18949=ORIENTED_EDGE ( 'NONE', *, *, #58159, .F. ) ;
#18950=DIRECTION ( 'NONE',  ( 0.000000000000000000, 0.000000000000000000, 1.000000000000000000 ) ) ;
#18951=EDGE_CURVE ( 'NONE', #40089, #122097, #65464, .T. ) ;
#18952=EDGE_CURVE ( 'NONE', #24264, #108022, #78092, .T. ) ;
#18953=CARTESIAN_POINT ( 'NONE',  ( -8.750000000000008882, 2.500000000000000000, -2.857883832488653741 ) ) ;
#18954=EDGE_CURVE ( 'NONE', #75945, #49108, #65841, .T. ) ;
#18955=FACE_BOUND ( 'NONE', #112932, .T. ) ;
#18956=ADVANCED_FACE ( 'NONE', ( #125418 ), #96581, .T. ) ;
#18957=DIRECTION ( 'NONE',  ( 0.000000000000000000, 0.000000000000000000, -1.000000000000000000 ) ) ;
#18959=DIRECTION ( 'NONE',  ( 0.000000000000000000, 0.000000000000000000, 1.000000000000000000 ) ) ;
#18960=EDGE_CURVE ( 'NONE', #108184, #62695, #53058, .T. ) ;
#18961=CIRCLE ( 'NONE', #92125, 0.1000000000000000472 ) ;
#18962=VECTOR ( 'NONE', #110831, 1000.000000000000000 ) ;
#18963=EDGE_LOOP ( 'NONE', ( #13628, #44121 ) ) ;
#18964=CARTESIAN_POINT ( 'NONE',  ( -2.700000000000030376, 12.50000000000000000, 3.983716857408420964 ) ) ;
#18965=AXIS2_PLACEMENT_3D ( 'NONE', #108399, #128046, #50147 ) ;
#18966=DIRECTION ( 'NONE',  ( 0.000000000000000000, 0.000000000000000000, 1.000000000000000000 ) ) ;
#18967=ADVANCED_FACE ( 'NONE', ( #24643 ), #76965, .T. ) ;
#18968=DIRECTION ( 'NONE',  ( 0.000000000000000000, 1.000000000000000000, 0.000000000000000000 ) ) ;
#18969=CARTESIAN_POINT ( 'NONE',  ( -5.000000000000024869, 2.500000000000000000, -5.122947341949753763 ) ) ;
#18970=ORIENTED_EDGE ( 'NONE', *, *, #105000, .F. ) ;
#18971=DIRECTION ( 'NONE',  ( 0.000000000000000000, 0.000000000000000000, -1.000000000000000000 ) ) ;
#18972=EDGE_CURVE ( 'NONE', #39660, #52720, #36349, .T. ) ;
#18973=AXIS2_PLACEMENT_3D ( 'NONE', #42651, #93021, #41987 ) ;
#18974=EDGE_CURVE ( 'NONE', #116295, #20224, #21664, .T. ) ;
#18976=ORIENTED_EDGE ( 'NONE', *, *, #22400, .T. ) ;
#18977=EDGE_LOOP ( 'NONE', ( #49172, #18652, #38149, #127878 ) ) ;
#18978=FACE_OUTER_BOUND ( 'NONE', #20022, .T. ) ;
#18979=DIRECTION ( 'NONE',  ( 0.000000000000000000, 0.000000000000000000, 1.000000000000000000 ) ) ;
#18980=FACE_BOUND ( 'NONE', #74132, .T. ) ;
#18981=ADVANCED_FACE ( 'NONE', ( #98513 ), #71838, .T. ) ;
#18982=FACE_OUTER_BOUND ( 'NONE', #10974, .T. ) ;
#18983=ORIENTED_EDGE ( 'NONE', *, *, #39539, .T. ) ;
#18984=DIRECTION ( 'NONE',  ( 0.000000000000000000, 0.000000000000000000, 1.000000000000000000 ) ) ;
#18985=ORIENTED_EDGE ( 'NONE', *, *, #96856, .T. ) ;
#18988=ORIENTED_EDGE ( 'NONE', *, *, #102493, .F. ) ;
#18989=CARTESIAN_POINT ( 'NONE',  ( -5.650000000000023448, 2.500000000000000000, -6.741600689897078169 ) ) ;
#18990=CARTESIAN_POINT ( 'NONE',  ( -6.250000000000021316, 12.50000000000000000, -1.472243186433550122 ) ) ;
#18991=AXIS2_PLACEMENT_3D ( 'NONE', #94214, #73930, #14349 ) ;
#18992=CARTESIAN_POINT ( 'NONE',  ( -11.05000000000000071, 2.500000000000000000, 6.841600689897072485 ) ) ;
#18993=CARTESIAN_POINT ( 'NONE',  ( 9.399999999999915090, 2.500000000000000000, -4.676537180435977881 ) ) ;
#18994=CIRCLE ( 'NONE', #42003, 0.09999999999999982514 ) ;
#18995=CIRCLE ( 'NONE', #92170, 0.09999999999999982514 ) ;
#18996=VERTEX_POINT ( 'NONE', #89991 ) ;
#18997=DIRECTION ( 'NONE',  ( 0.000000000000000000, 0.000000000000000000, 1.000000000000000000 ) ) ;
#18998=CARTESIAN_POINT ( 'NONE',  ( 9.399999999999918643, 12.50000000000000000, -0.3464101615137782364 ) ) ;
#18999=DIRECTION ( 'NONE',  ( 0.000000000000000000, 0.000000000000000000, 1.000000000000000000 ) ) ;
#19000=CARTESIAN_POINT ( 'NONE',  ( -1.850000000000033840, 12.50000000000000000, 1.818653347947321475 ) ) ;
#19001=ORIENTED_EDGE ( 'NONE', *, *, #68878, .T. ) ;
#19002=ORIENTED_EDGE ( 'NONE', *, *, #41938, .F. ) ;
#19003=DIRECTION ( 'NONE',  ( 0.000000000000000000, -0.9999939076577903929, 0.003490651415223739937 ) ) ;
#19004=AXIS2_PLACEMENT_3D ( 'NONE', #72846, #12620, #22479 ) ;
#19005=ORIENTED_EDGE ( 'NONE', *, *, #12472, .F. ) ;
#19006=CARTESIAN_POINT ( 'NONE',  ( 9.399999999999918643, 12.50000000000000000, 0.3464101615137736845 ) ) ;
#19007=AXIS2_PLACEMENT_3D ( 'NONE', #120498, #70751, #20998 ) ;
#19008=CARTESIAN_POINT ( 'NONE',  ( 17.50000000000000000, -2.499999999999999556, -2.666666666666662522 ) ) ;
#19009=EDGE_CURVE ( 'NONE', #56486, #24243, #59928, .T. ) ;
#19010=FACE_OUTER_BOUND ( 'NONE', #12861, .T. ) ;
#19011=CARTESIAN_POINT ( 'NONE',  ( -12.89999999999999325, 2.500000000000000000, 0.6928203230275535862 ) ) ;
#19012=EDGE_LOOP ( 'NONE', ( #11790, #52183, #39715, #35882 ) ) ;
#19013=DIRECTION ( 'NONE',  ( 0.000000000000000000, 1.000000000000000000, 0.000000000000000000 ) ) ;
#19014=EDGE_CURVE ( 'NONE', #6037, #94991, #17429, .T. ) ;
#19015=CARTESIAN_POINT ( 'NONE',  ( -12.69999999999999218, 2.500000000000000000, 4.676537180435972552 ) ) ;
#19016=DIRECTION ( 'NONE',  ( 0.000000000000000000, 1.000000000000000000, 0.000000000000000000 ) ) ;
#19018=CARTESIAN_POINT ( 'NONE',  ( 6.699999999999930012, 12.50000000000000000, 4.330127018922196314 ) ) ;
#19019=FACE_OUTER_BOUND ( 'NONE', #17913, .T. ) ;
#19020=EDGE_LOOP ( 'NONE', ( #79457, #98309 ) ) ;
#19021=AXIS2_PLACEMENT_3D ( 'NONE', #108478, #128134, #98012 ) ;
#19022=ORIENTED_EDGE ( 'NONE', *, *, #3044, .T. ) ;
#19023=CARTESIAN_POINT ( 'NONE',  ( -12.69999999999999396, 12.50000000000000000, 0.3464101615137776813 ) ) ;
#19024=ORIENTED_EDGE ( 'NONE', *, *, #59632, .T. ) ;
#19025=LINE ( 'NONE', #58974, #105726 ) ;
#19027=EDGE_LOOP ( 'NONE', ( #97000, #54917 ) ) ;
#19028=EDGE_LOOP ( 'NONE', ( #25520, #70327 ) ) ;
#19029=FACE_OUTER_BOUND ( 'NONE', #16467, .T. ) ;
#19030=AXIS2_PLACEMENT_3D ( 'NONE', #84817, #45560, #95295 ) ;
#19031=DIRECTION ( 'NONE',  ( 0.000000000000000000, -0.9999939076577903929, 0.003490651415223739937 ) ) ;
#19032=DIRECTION ( 'NONE',  ( 0.000000000000000000, -0.000000000000000000, 1.000000000000000000 ) ) ;
#19033=LINE ( 'NONE', #70732, #74478 ) ;
#19034=CONICAL_SURFACE ( 'NONE', #117224, 0.1000000000000002554, 0.003490658503988666988 ) ;
#19035=AXIS2_PLACEMENT_3D ( 'NONE', #42424, #82353, #32625 ) ;
#19036=DIRECTION ( 'NONE',  ( -0.000000000000000000, -1.000000000000000000, -0.000000000000000000 ) ) ;
#19037=DIRECTION ( 'NONE',  ( -4.274815082592931898E-19, -0.9999939076577903929, -0.003490651415223739937 ) ) ;
#19038=DIRECTION ( 'NONE',  ( 0.000000000000000000, 0.000000000000000000, 1.000000000000000000 ) ) ;
#19039=CARTESIAN_POINT ( 'NONE',  ( 10.39999999999991154, 2.500000000000000000, 5.022947341949748790 ) ) ;
#19040=VERTEX_POINT ( 'NONE', #99191 ) ;
#19041=ORIENTED_EDGE ( 'NONE', *, *, #49397, .T. ) ;
#19042=DIRECTION ( 'NONE',  ( 0.000000000000000000, 0.000000000000000000, -1.000000000000000000 ) ) ;
#19043=ORIENTED_EDGE ( 'NONE', *, *, #59802, .T. ) ;
#19044=VERTEX_POINT ( 'NONE', #108977 ) ;
#19045=DIRECTION ( 'NONE',  ( -0.000000000000000000, -1.000000000000000000, -0.000000000000000000 ) ) ;
#19046=EDGE_CURVE ( 'NONE', #60091, #57903, #27862, .T. ) ;
#19047=FACE_OUTER_BOUND ( 'NONE', #61451, .T. ) ;
#19048=CARTESIAN_POINT ( 'NONE',  ( -2.900000000000029665, 12.50000000000000000, 3.637306695894644726 ) ) ;
#19049=DIRECTION ( 'NONE',  ( 0.000000000000000000, 0.000000000000000000, 1.000000000000000000 ) ) ;
#19050=AXIS2_PLACEMENT_3D ( 'NONE', #34047, #92310, #84430 ) ;
#19051=CARTESIAN_POINT ( 'NONE',  ( -4.600000000000024514, 2.500000000000000000, 3.737306695894644371 ) ) ;
#19052=ORIENTED_EDGE ( 'NONE', *, *, #83850, .F. ) ;
#19053=CONICAL_SURFACE ( 'NONE', #104828, 0.09999999999999999167, 0.003490658503988666988 ) ;
#19054=ORIENTED_EDGE ( 'NONE', *, *, #44438, .T. ) ;
#19055=CARTESIAN_POINT ( 'NONE',  ( 5.399999999999936406, 2.500000000000000000, -5.022947341949754119 ) ) ;
#19056=AXIS2_PLACEMENT_3D ( 'NONE', #75297, #68055, #115194 ) ;
#19057=ORIENTED_EDGE ( 'NONE', *, *, #61655, .T. ) ;
#19058=CARTESIAN_POINT ( 'NONE',  ( 6.049999999999934097, 2.500000000000000000, 6.148780366869520897 ) ) ;
#19059=ORIENTED_EDGE ( 'NONE', *, *, #48590, .F. ) ;
#19060=AXIS2_PLACEMENT_3D ( 'NONE', #19873, #59826, #67010 ) ;
#19061=ADVANCED_FACE ( 'NONE', ( #59282 ), #79547, .T. ) ;
#19062=ADVANCED_FACE ( 'NONE', ( #80195 ), #38343, .T. ) ;
#19063=ORIENTED_EDGE ( 'NONE', *, *, #107956, .F. ) ;
#19064=DIRECTION ( 'NONE',  ( 0.000000000000000000, 0.000000000000000000, 1.000000000000000000 ) ) ;
#19065=DIRECTION ( 'NONE',  ( 0.000000000000000000, 0.000000000000000000, -1.000000000000000000 ) ) ;
#19066=DIRECTION ( 'NONE',  ( 0.000000000000000000, 1.000000000000000000, 0.000000000000000000 ) ) ;
#19067=CARTESIAN_POINT ( 'NONE',  ( 3.549999999999944755, 2.500000000000000000, -6.841600689897077814 ) ) ;
#19069=LINE ( 'NONE', #46614, #61695 ) ;
#19070=ORIENTED_EDGE ( 'NONE', *, *, #28557, .F. ) ;
#19071=CARTESIAN_POINT ( 'NONE',  ( -0.8500000000000386136, 2.500000000000000000, 7.088010851410848190 ) ) ;
#19072=LINE ( 'NONE', #78680, #28600 ) ;
#19073=EDGE_CURVE ( 'NONE', #125678, #72018, #13231, .T. ) ;
#19074=LINE ( 'NONE', #38770, #62551 ) ;
#19075=PLANE ( 'NONE',  #15857 ) ;
#19076=CARTESIAN_POINT ( 'NONE',  ( 1.899999999999949507, 2.500000000000000000, 3.983716857408420964 ) ) ;
#19077=ORIENTED_EDGE ( 'NONE', *, *, #62084, .F. ) ;
#19078=ORIENTED_EDGE ( 'NONE', *, *, #116288, .T. ) ;
#19079=DIRECTION ( 'NONE',  ( 0.000000000000000000, 0.000000000000000000, 1.000000000000000000 ) ) ;
#19080=ORIENTED_EDGE ( 'NONE', *, *, #94206, .F. ) ;
#19081=DIRECTION ( 'NONE',  ( 0.000000000000000000, 0.000000000000000000, 1.000000000000000000 ) ) ;
#19082=DIRECTION ( 'NONE',  ( 0.000000000000000000, 1.000000000000000000, 0.000000000000000000 ) ) ;
#19083=CIRCLE ( 'NONE', #79750, 0.06509327318403745899 ) ;
#19084=VERTEX_POINT ( 'NONE', #110287 ) ;
#19085=DIRECTION ( 'NONE',  ( 0.000000000000000000, 0.000000000000000000, 1.000000000000000000 ) ) ;
#19086=DIRECTION ( 'NONE',  ( -0.000000000000000000, -1.000000000000000000, -0.000000000000000000 ) ) ;
#19088=CARTESIAN_POINT ( 'NONE',  ( 5.399999999999935518, 2.500000000000000000, -4.230127018922201998 ) ) ;
#19089=ORIENTED_EDGE ( 'NONE', *, *, #114552, .F. ) ;
#19090=AXIS2_PLACEMENT_3D ( 'NONE', #90261, #39911, #37958 ) ;
#19091=EDGE_CURVE ( 'NONE', #53683, #107604, #38404, .T. ) ;
#19092=CARTESIAN_POINT ( 'NONE',  ( -2.300000000000033129, 2.500000000000000000, 4.083716857408420609 ) ) ;
#19093=ORIENTED_EDGE ( 'NONE', *, *, #31860, .T. ) ;
#19094=EDGE_CURVE ( 'NONE', #97989, #106677, #78272, .T. ) ;
#19095=CARTESIAN_POINT ( 'NONE',  ( 4.399999999999937295, 2.500000000000000000, 4.676537180435972552 ) ) ;
#19096=DIRECTION ( 'NONE',  ( 0.000000000000000000, 0.000000000000000000, -1.000000000000000000 ) ) ;
#19097=EDGE_CURVE ( 'NONE', #84309, #89637, #97242, .T. ) ;
#19098=DIRECTION ( 'NONE',  ( 0.000000000000000000, 0.000000000000000000, 1.000000000000000000 ) ) ;
#19099=CIRCLE ( 'NONE', #23231, 0.1000000000000002554 ) ;
#19101=EDGE_LOOP ( 'NONE', ( #29070, #122977, #50999, #2205 ) ) ;
#19102=CARTESIAN_POINT ( 'NONE',  ( 3.349999999999944578, 2.500000000000000000, -5.702370205355749455 ) ) ;
#19103=AXIS2_PLACEMENT_3D ( 'NONE', #74974, #55966, #15383 ) ;
#19104=EDGE_CURVE ( 'NONE', #77225, #1350, #23723, .T. ) ;
#19105=EDGE_CURVE ( 'NONE', #10534, #14739, #32145, .T. ) ;
#19106=VERTEX_POINT ( 'NONE', #19316 ) ;
#19107=DIRECTION ( 'NONE',  ( 0.000000000000000000, 0.000000000000000000, 1.000000000000000000 ) ) ;
#19108=DIRECTION ( 'NONE',  ( 0.000000000000000000, 0.000000000000000000, 1.000000000000000000 ) ) ;
#19109=ADVANCED_FACE ( 'NONE', ( #128675 ), #69675, .T. ) ;
#19110=CONICAL_SURFACE ( 'NONE', #94432, 0.1000000000000000472, 0.003490658503988666988 ) ;
#19111=FACE_OUTER_BOUND ( 'NONE', #80237, .T. ) ;
#19112=ORIENTED_EDGE ( 'NONE', *, *, #116504, .F. ) ;
#19113=DIRECTION ( 'NONE',  ( 0.000000000000000000, 0.000000000000000000, 1.000000000000000000 ) ) ;
#19114=ADVANCED_FACE ( 'NONE', ( #39008 ), #90598, .T. ) ;
#19115=DIRECTION ( 'NONE',  ( 0.000000000000000000, 1.000000000000000000, 0.000000000000000000 ) ) ;
#19116=CIRCLE ( 'NONE', #109008, 0.1000000000000002554 ) ;
#19117=CIRCLE ( 'NONE', #48392, 0.06509327318403745899 ) ;
#19119=CARTESIAN_POINT ( 'NONE',  ( -8.350000000000013856, 2.500000000000000000, -7.188010851410848723 ) ) ;
#19120=EDGE_LOOP ( 'NONE', ( #43335, #59011, #69081, #20477 ) ) ;
#19121=ADVANCED_FACE ( 'NONE', ( #9514 ), #9135, .T. ) ;
#19122=DIRECTION ( 'NONE',  ( 0.000000000000000000, 0.000000000000000000, 1.000000000000000000 ) ) ;
#19123=ORIENTED_EDGE ( 'NONE', *, *, #103812, .F. ) ;
#19124=FACE_OUTER_BOUND ( 'NONE', #85159, .T. ) ;
#19125=PLANE ( 'NONE',  #49998 ) ;
#19127=VERTEX_POINT ( 'NONE', #80841 ) ;
#19128=CARTESIAN_POINT ( 'NONE',  ( -7.050000000000016698, 2.500000000000000000, -6.595190528383302109 ) ) ;
#19129=DIRECTION ( 'NONE',  ( -0.000000000000000000, -1.000000000000000000, -0.000000000000000000 ) ) ;
#19130=ORIENTED_EDGE ( 'NONE', *, *, #111194, .T. ) ;
#19132=PLANE ( 'NONE',  #1177 ) ;
#19133=DIRECTION ( 'NONE',  ( -0.000000000000000000, -1.000000000000000000, -0.000000000000000000 ) ) ;
#19134=VECTOR ( 'NONE', #22225, 1000.000000000000000 ) ;
#19136=CARTESIAN_POINT ( 'NONE',  ( -4.600000000000028955, 2.500000000000000000, -4.230127018922201998 ) ) ;
#19137=VECTOR ( 'NONE', #95398, 1000.000000000000000 ) ;
#19138=AXIS2_PLACEMENT_3D ( 'NONE', #23097, #124530, #103602 ) ;
#19139=LINE ( 'NONE', #97082, #41076 ) ;
#19140=DIRECTION ( 'NONE',  ( 0.000000000000000000, 0.000000000000000000, -1.000000000000000000 ) ) ;
#19141=CONICAL_SURFACE ( 'NONE', #90252, 0.09999999999999982514, 0.003490658503988666988 ) ;
#19142=ORIENTED_EDGE ( 'NONE', *, *, #104767, .F. ) ;
#19143=AXIS2_PLACEMENT_3D ( 'NONE', #81515, #99869, #10194 ) ;
#19144=ORIENTED_EDGE ( 'NONE', *, *, #110163, .F. ) ;
#19145=VERTEX_POINT ( 'NONE', #23188 ) ;
#19146=VERTEX_POINT ( 'NONE', #101115 ) ;
#19147=CARTESIAN_POINT ( 'NONE',  ( 14.54999999999989591, 2.500000000000000000, 2.065063509461097624 ) ) ;
#19148=DIRECTION ( 'NONE',  ( 0.000000000000000000, -0.000000000000000000, 1.000000000000000000 ) ) ;
#19149=VECTOR ( 'NONE', #80216, 1000.000000000000000 ) ;
#19150=DIRECTION ( 'NONE',  ( 0.000000000000000000, 1.000000000000000000, 0.000000000000000000 ) ) ;
#19151=ORIENTED_EDGE ( 'NONE', *, *, #43972, .T. ) ;
#19152=FACE_BOUND ( 'NONE', #75832, .T. ) ;
#19153=ORIENTED_EDGE ( 'NONE', *, *, #56398, .F. ) ;
#19154=CARTESIAN_POINT ( 'NONE',  ( -5.000000000000022204, 2.500000000000000000, -0.7928203230275542301 ) ) ;
#19155=PLANE ( 'NONE',  #5987 ) ;
#19156=AXIS2_PLACEMENT_3D ( 'NONE', #62000, #22081, #52807 ) ;
#19157=CARTESIAN_POINT ( 'NONE',  ( 7.499999999999925393, 12.50000000000000000, -3.637306695894650055 ) ) ;
#19158=EDGE_CURVE ( 'NONE', #12823, #31364, #115732, .T. ) ;
#19159=DIRECTION ( 'NONE',  ( 0.000000000000000000, 0.000000000000000000, 1.000000000000000000 ) ) ;
#19160=CARTESIAN_POINT ( 'NONE',  ( 1.649999999999949729, 2.500000000000000000, 5.702370205355745014 ) ) ;
#19162=DIRECTION ( 'NONE',  ( -0.000000000000000000, 1.000000000000000000, -0.000000000000000000 ) ) ;
#19163=CARTESIAN_POINT ( 'NONE',  ( 14.14999999999989733, 12.50000000000000000, 1.537336459617582918 ) ) ;
#19164=CARTESIAN_POINT ( 'NONE',  ( -7.300000000000018474, 2.500000000000000000, 0.4464101615137735513 ) ) ;
#19165=DIRECTION ( 'NONE',  ( 0.000000000000000000, 0.000000000000000000, 1.000000000000000000 ) ) ;
#19166=EDGE_CURVE ( 'NONE', #87864, #69735, #59338, .T. ) ;
#19167=EDGE_LOOP ( 'NONE', ( #69551, #93479 ) ) ;
#19168=ORIENTED_EDGE ( 'NONE', *, *, #74978, .T. ) ;
#19169=ORIENTED_EDGE ( 'NONE', *, *, #102173, .T. ) ;
#19170=ORIENTED_EDGE ( 'NONE', *, *, #19073, .F. ) ;
#19171=CARTESIAN_POINT ( 'NONE',  ( 16.89179977596573323, -0.9177129796144657403, -5.694535519821270597 ) ) ;
#19172=CARTESIAN_POINT ( 'NONE',  ( -12.09999999999999609, 12.50000000000000000, 1.734723475976807094E-15 ) ) ;
#19174=ORIENTED_EDGE ( 'NONE', *, *, #61461, .F. ) ;
#19175=EDGE_LOOP ( 'NONE', ( #26062, #113461 ) ) ;
#19176=VERTEX_POINT ( 'NONE', #52648 ) ;
#19177=DIRECTION ( 'NONE',  ( 0.000000000000000000, 0.000000000000000000, 1.000000000000000000 ) ) ;
#19178=CIRCLE ( 'NONE', #29670, 0.06509327318403741736 ) ;
#19179=CONICAL_SURFACE ( 'NONE', #92348, 0.1000000000000002554, 0.003490658503988666988 ) ;
#19180=DIRECTION ( 'NONE',  ( 0.000000000000000000, -0.9999939076577903929, 0.003490651415223739937 ) ) ;
#19181=CARTESIAN_POINT ( 'NONE',  ( -6.250000000000015987, 12.50000000000000000, 5.802370205355744659 ) ) ;
#19182=CARTESIAN_POINT ( 'NONE',  ( -9.600000000000008527, 2.500000000000000000, -5.022947341949749678 ) ) ;
#19183=CARTESIAN_POINT ( 'NONE',  ( 3.749999999999940492, 12.50000000000000000, 5.802370205355744659 ) ) ;
#19184=CARTESIAN_POINT ( 'NONE',  ( 11.84999999999990372, 2.500000000000000000, -6.248780366869526759 ) ) ;
#19185=CARTESIAN_POINT ( 'NONE',  ( -15.59999999999998010, 2.500000000000000000, -0.4464101615137759382 ) ) ;
#19186=ORIENTED_EDGE ( 'NONE', *, *, #80038, .F. ) ;
#19187=CIRCLE ( 'NONE', #117461, 0.1000000000000002554 ) ;
#19188=CONICAL_SURFACE ( 'NONE', #8724, 0.1000000000000002554, 0.003490658503988666988 ) ;
#19189=CARTESIAN_POINT ( 'NONE',  ( 11.84999999999990372, 12.50000000000000000, 2.511473670974873507 ) ) ;
#19190=EDGE_LOOP ( 'NONE', ( #59348, #47705, #77584, #95564 ) ) ;
#19191=CIRCLE ( 'NONE', #92357, 0.09999999999999982514 ) ;
#19192=EDGE_LOOP ( 'NONE', ( #100633, #36353 ) ) ;
#19193=CIRCLE ( 'NONE', #12934, 0.06509327318403745899 ) ;
#19194=ORIENTED_EDGE ( 'NONE', *, *, #107649, .T. ) ;
#19195=VECTOR ( 'NONE', #52506, 1000.000000000000000 ) ;
#19196=CARTESIAN_POINT ( 'NONE',  ( -0.4500000000000402012, 12.50000000000000000, 6.495190528383297135 ) ) ;
#19198=VERTEX_POINT ( 'NONE', #121392 ) ;
#19199=ORIENTED_EDGE ( 'NONE', *, *, #70323, .T. ) ;
#19200=CONICAL_SURFACE ( 'NONE', #46307, 0.09999999999999999167, 0.003490658503988666988 ) ;
#19201=DIRECTION ( 'NONE',  ( 0.000000000000000000, 0.000000000000000000, 1.000000000000000000 ) ) ;
#19202=CONICAL_SURFACE ( 'NONE', #58940, 0.1000000000000002554, 0.003490658503988666988 ) ;
#19203=EDGE_CURVE ( 'NONE', #100401, #20290, #2250, .T. ) ;
#19204=CARTESIAN_POINT ( 'NONE',  ( -2.900000000000029665, 12.50000000000000000, 4.395220292106234439 ) ) ;
#19206=CARTESIAN_POINT ( 'NONE',  ( -1.650000000000034328, 2.500000000000000000, -7.188010851410854052 ) ) ;
#19207=VECTOR ( 'NONE', #74861, 1000.000000000000000 ) ;
#19208=AXIS2_PLACEMENT_3D ( 'NONE', #44663, #114051, #63668 ) ;
#19209=CIRCLE ( 'NONE', #115642, 0.06509327318403745899 ) ;
#19211=CONICAL_SURFACE ( 'NONE', #65279, 0.1000000000000000472, 0.003490658503988666988 ) ;
#19212=ORIENTED_EDGE ( 'NONE', *, *, #95301, .T. ) ;
#19213=DIRECTION ( 'NONE',  ( -0.000000000000000000, 1.000000000000000000, -0.000000000000000000 ) ) ;
#19214=EDGE_CURVE ( 'NONE', #60736, #124494, #122686, .T. ) ;
#19215=EDGE_LOOP ( 'NONE', ( #82591, #124154 ) ) ;
#19216=DIRECTION ( 'NONE',  ( 0.000000000000000000, 0.000000000000000000, -1.000000000000000000 ) ) ;
#19217=ORIENTED_EDGE ( 'NONE', *, *, #87183, .T. ) ;
#19218=CARTESIAN_POINT ( 'NONE',  ( 5.849999999999934808, 2.500000000000000000, -5.802370205355749988 ) ) ;
#19219=AXIS2_PLACEMENT_3D ( 'NONE', #86449, #53776, #85804 ) ;
#19220=DIRECTION ( 'NONE',  ( 0.000000000000000000, 0.000000000000000000, -1.000000000000000000 ) ) ;
#19221=ORIENTED_EDGE ( 'NONE', *, *, #42360, .F. ) ;
#19223=EDGE_CURVE ( 'NONE', #52767, #20628, #110917, .T. ) ;
#19224=DIRECTION ( 'NONE',  ( 0.000000000000000000, -0.9999939076577903929, 0.003490651415223739937 ) ) ;
#19225=EDGE_CURVE ( 'NONE', #88967, #112846, #92585, .T. ) ;
#19226=ORIENTED_EDGE ( 'NONE', *, *, #120792, .T. ) ;
#19227=EDGE_CURVE ( 'NONE', #81889, #55268, #123333, .T. ) ;
#19228=FACE_OUTER_BOUND ( 'NONE', #4870, .T. ) ;
#19229=ORIENTED_EDGE ( 'NONE', *, *, #127851, .F. ) ;
#19230=VERTEX_POINT ( 'NONE', #51392 ) ;
#19231=DIRECTION ( 'NONE',  ( 0.000000000000000000, 0.000000000000000000, 1.000000000000000000 ) ) ;
#19232=DIRECTION ( 'NONE',  ( 0.000000000000000000, 0.000000000000000000, 1.000000000000000000 ) ) ;
#19233=EDGE_CURVE ( 'NONE', #77871, #15508, #82118, .T. ) ;
#19234=FACE_OUTER_BOUND ( 'NONE', #1926, .T. ) ;
#19235=DIRECTION ( 'NONE',  ( 0.000000000000000000, 1.000000000000000000, 0.000000000000000000 ) ) ;
#19236=LINE ( 'NONE', #248, #116840 ) ;
#19237=ORIENTED_EDGE ( 'NONE', *, *, #2018, .F. ) ;
#19238=CARTESIAN_POINT ( 'NONE',  ( -4.150000000000025224, 2.500000000000000000, 2.757883832488649656 ) ) ;
#19239=CIRCLE ( 'NONE', #123784, 0.06509327318403745899 ) ;
#19240=AXIS2_PLACEMENT_3D ( 'NONE', #122439, #35346, #13745 ) ;
#19241=ORIENTED_EDGE ( 'NONE', *, *, #20031, .F. ) ;
#19242=CARTESIAN_POINT ( 'NONE',  ( -3.550000000000028244, 12.50000000000000000, -1.883746621131363597 ) ) ;
#19243=CARTESIAN_POINT ( 'NONE',  ( 7.949999999999922018, 12.50000000000000000, -2.230156782645139391 ) ) ;
#19244=AXIS2_PLACEMENT_3D ( 'NONE', #55206, #54531, #4782 ) ;
#19245=CIRCLE ( 'NONE', #92412, 0.1000000000000000472 ) ;
#19246=CIRCLE ( 'NONE', #113340, 0.06509327318403745899 ) ;
#19247=AXIS2_PLACEMENT_3D ( 'NONE', #97113, #29036, #27720 ) ;
#19248=AXIS2_PLACEMENT_3D ( 'NONE', #127157, #117284, #55186 ) ;
#19249=CARTESIAN_POINT ( 'NONE',  ( 0.1999999999999636513, 2.500000000000000000, -0.2464101615137760659 ) ) ;
#19250=DIRECTION ( 'NONE',  ( 0.000000000000000000, 1.000000000000000000, 0.000000000000000000 ) ) ;
#19251=LINE ( 'NONE', #59215, #63205 ) ;
#19252=DIRECTION ( 'NONE',  ( 0.000000000000000000, 1.000000000000000000, 0.000000000000000000 ) ) ;
#19253=DIRECTION ( 'NONE',  ( 0.000000000000000000, 0.000000000000000000, 1.000000000000000000 ) ) ;
#19254=ORIENTED_EDGE ( 'NONE', *, *, #57822, .T. ) ;
#19255=AXIS2_PLACEMENT_3D ( 'NONE', #84924, #16798, #44349 ) ;
#19257=DIRECTION ( 'NONE',  ( 0.000000000000000000, -0.9999939076577903929, 0.003490651415223739937 ) ) ;
#19259=ORIENTED_EDGE ( 'NONE', *, *, #18960, .F. ) ;
#19260=EDGE_CURVE ( 'NONE', #84685, #14124, #25863, .T. ) ;
#19261=DIRECTION ( 'NONE',  ( 0.000000000000000000, -0.9999939076577903929, 0.003490651415223739937 ) ) ;
#19262=ORIENTED_EDGE ( 'NONE', *, *, #75531, .F. ) ;
#19264=CARTESIAN_POINT ( 'NONE',  ( -12.94999999999999218, 2.500000000000000000, -2.265063509461099578 ) ) ;
#19265=EDGE_CURVE ( 'NONE', #107104, #14028, #50911, .T. ) ;
#19266=EDGE_CURVE ( 'NONE', #57219, #114003, #126111, .T. ) ;
#19267=VERTEX_POINT ( 'NONE', #42870 ) ;
#19268=CARTESIAN_POINT ( 'NONE',  ( 7.699999999999923794, 2.500000000000000000, -0.3464101615137783474 ) ) ;
#19269=CARTESIAN_POINT ( 'NONE',  ( -7.900000000000014566, 2.500000000000000000, 0.5928203230275495006 ) ) ;
#19270=EDGE_CURVE ( 'NONE', #54425, #41455, #41572, .T. ) ;
#19271=EDGE_CURVE ( 'NONE', #113210, #19759, #109483, .T. ) ;
#19273=VERTEX_POINT ( 'NONE', #31731 ) ;
#19274=CARTESIAN_POINT ( 'NONE',  ( 8.949999999999921130, 12.50000000000000000, -6.841600689897078702 ) ) ;
#19276=CARTESIAN_POINT ( 'NONE',  ( 4.599999999999935696, 2.500000000000000000, 4.922947341949748257 ) ) ;
#19277=ORIENTED_EDGE ( 'NONE', *, *, #13971, .T. ) ;
#19278=CARTESIAN_POINT ( 'NONE',  ( 13.94999999999989804, 2.500000000000000000, 1.818653347947321475 ) ) ;
#19279=DIRECTION ( 'NONE',  ( 0.000000000000000000, 1.000000000000000000, 0.000000000000000000 ) ) ;
#19280=CIRCLE ( 'NONE', #107113, 0.09999999999999999167 ) ;
#19281=ORIENTED_EDGE ( 'NONE', *, *, #120745, .T. ) ;
#19282=AXIS2_PLACEMENT_3D ( 'NONE', #128565, #66386, #76861 ) ;
#19283=ADVANCED_FACE ( 'NONE', ( #22578 ), #46697, .T. ) ;
#19284=CIRCLE ( 'NONE', #44436, 0.06509327318403741736 ) ;
#19285=EDGE_CURVE ( 'NONE', #95487, #79569, #86393, .T. ) ;
#19286=CONICAL_SURFACE ( 'NONE', #6749, 0.1000000000000002554, 0.003490658503988666988 ) ;
#19287=ORIENTED_EDGE ( 'NONE', *, *, #101124, .F. ) ;
#19288=ORIENTED_EDGE ( 'NONE', *, *, #123934, .T. ) ;
#19289=CARTESIAN_POINT ( 'NONE',  ( 9.799999999999913669, 2.500000000000000000, 4.576537180435972019 ) ) ;
#19290=DIRECTION ( 'NONE',  ( 0.000000000000000000, 0.000000000000000000, -1.000000000000000000 ) ) ;
#19291=CARTESIAN_POINT ( 'NONE',  ( 5.199999999999931788, 2.500000000000000000, 4.576537180435972019 ) ) ;
#19292=FACE_BOUND ( 'NONE', #113965, .T. ) ;
#19293=ORIENTED_EDGE ( 'NONE', *, *, #13608, .T. ) ;
#19294=DIRECTION ( 'NONE',  ( -4.274815082592931898E-19, -0.9999939076577903929, -0.003490651415223739937 ) ) ;
#19295=DIRECTION ( 'NONE',  ( 0.000000000000000000, 0.000000000000000000, -1.000000000000000000 ) ) ;
#19296=CONICAL_SURFACE ( 'NONE', #17125, 0.1000000000000000472, 0.003490658503988666988 ) ;
#19297=ORIENTED_EDGE ( 'NONE', *, *, #94333, .F. ) ;
#19298=DIRECTION ( 'NONE',  ( 0.000000000000000000, -0.9999939076577903929, 0.003490651415223739937 ) ) ;
#19299=CARTESIAN_POINT ( 'NONE',  ( 17.45652781226509731, 2.453230724138542485, 4.494708854620872884 ) ) ;
#19300=CIRCLE ( 'NONE', #79953, 0.06509327318403745899 ) ;
#19301=CIRCLE ( 'NONE', #123860, 0.1000000000000002554 ) ;
#19302=AXIS2_PLACEMENT_3D ( 'NONE', #7265, #86479, #47216 ) ;
#19303=DIRECTION ( 'NONE',  ( -4.274815082592931898E-19, -0.9999939076577903929, -0.003490651415223739937 ) ) ;
#19304=CARTESIAN_POINT ( 'NONE',  ( -6.900000000000019007, 12.50000000000000000, -3.983716857408426293 ) ) ;
#19305=CARTESIAN_POINT ( 'NONE',  ( -8.350000000000012079, 2.500000000000000000, -2.957883832488653830 ) ) ;
#19306=DIRECTION ( 'NONE',  ( 0.000000000000000000, 0.000000000000000000, 1.000000000000000000 ) ) ;
#19307=VECTOR ( 'NONE', #62161, 1000.000000000000000 ) ;
#19308=DIRECTION ( 'NONE',  ( 0.000000000000000000, 0.000000000000000000, -1.000000000000000000 ) ) ;
#19309=VERTEX_POINT ( 'NONE', #3556 ) ;
#19310=AXIS2_PLACEMENT_3D ( 'NONE', #45748, #46369, #33367 ) ;
#19311=ORIENTED_EDGE ( 'NONE', *, *, #30963, .T. ) ;
#19312=ORIENTED_EDGE ( 'NONE', *, *, #118379, .F. ) ;
#19313=ORIENTED_EDGE ( 'NONE', *, *, #67618, .T. ) ;
#19314=ORIENTED_EDGE ( 'NONE', *, *, #103584, .T. ) ;
#19315=CARTESIAN_POINT ( 'NONE',  ( -8.350000000000008527, 2.500000000000000000, 5.702370205355745014 ) ) ;
#19316=CARTESIAN_POINT ( 'NONE',  ( -10.65000000000000391, 2.500000000000000000, -1.918653347947322230 ) ) ;
#19317=ORIENTED_EDGE ( 'NONE', *, *, #16120, .F. ) ;
#19318=FACE_BOUND ( 'NONE', #71941, .T. ) ;
#19319=CARTESIAN_POINT ( 'NONE',  ( 7.099999999999927702, 2.500000000000000000, -3.537306695894649966 ) ) ;
#19320=DIRECTION ( 'NONE',  ( 0.000000000000000000, 1.000000000000000000, 0.000000000000000000 ) ) ;
#19321=CARTESIAN_POINT ( 'NONE',  ( 2.299999999999948752, 12.50000000000000000, -3.983716857408426293 ) ) ;
#19322=FACE_OUTER_BOUND ( 'NONE', #85181, .T. ) ;
#19323=CARTESIAN_POINT ( 'NONE',  ( -4.400000000000025224, 2.500000000000000000, 3.983716857408420076 ) ) ;
#19324=AXIS2_PLACEMENT_3D ( 'NONE', #18447, #68834, #108749 ) ;
#19325=CARTESIAN_POINT ( 'NONE',  ( 0.3999999999999555023, 2.500000000000000000, 4.330127018922196314 ) ) ;
#19327=ORIENTED_EDGE ( 'NONE', *, *, #67334, .T. ) ;
#19328=EDGE_CURVE ( 'NONE', #24109, #71913, #32406, .T. ) ;
#19329=EDGE_LOOP ( 'NONE', ( #82085, #28850 ) ) ;
#19330=AXIS2_PLACEMENT_3D ( 'NONE', #46195, #75644, #17360 ) ;
#19331=EDGE_LOOP ( 'NONE', ( #43766, #98215 ) ) ;
#19332=CONICAL_SURFACE ( 'NONE', #29819, 0.1000000000000000472, 0.003490658503988666988 ) ;
#19333=VECTOR ( 'NONE', #17616, 1000.000000000000000 ) ;
#19334=CARTESIAN_POINT ( 'NONE',  ( 10.84999999999990905, 12.50000000000000000, -6.495190528383302464 ) ) ;
#19335=DIRECTION ( 'NONE',  ( 0.000000000000000000, 1.000000000000000000, 0.000000000000000000 ) ) ;
#19336=ORIENTED_EDGE ( 'NONE', *, *, #106012, .F. ) ;
#19337=DIRECTION ( 'NONE',  ( 0.000000000000000000, 0.000000000000000000, -1.000000000000000000 ) ) ;
#19338=LINE ( 'NONE', #27233, #17728 ) ;
#19339=CIRCLE ( 'NONE', #113442, 0.06509327318403745899 ) ;
#19340=CIRCLE ( 'NONE', #40297, 0.06509327318403745899 ) ;
#19341=CIRCLE ( 'NONE', #15117, 0.06509327318403745899 ) ;
#19342=CARTESIAN_POINT ( 'NONE',  ( -4.200000000000025935, 12.50000000000000000, 4.265033745738159077 ) ) ;
#19344=DIRECTION ( 'NONE',  ( 0.000000000000000000, 0.000000000000000000, -1.000000000000000000 ) ) ;
#19345=CARTESIAN_POINT ( 'NONE',  ( 11.04999999999990656, 12.50000000000000000, -6.148780366869526226 ) ) ;
#19346=CIRCLE ( 'NONE', #71684, 0.06509327318403745899 ) ;
#19347=FACE_OUTER_BOUND ( 'NONE', #110322, .T. ) ;
#19348=VERTEX_POINT ( 'NONE', #123964 ) ;
#19349=CARTESIAN_POINT ( 'NONE',  ( -1.050000000000037348, 2.500000000000000000, -6.841600689897078702 ) ) ;
#19350=CIRCLE ( 'NONE', #54958, 0.06509327318403745899 ) ;
#19351=ORIENTED_EDGE ( 'NONE', *, *, #63764, .F. ) ;
#19352=ORIENTED_EDGE ( 'NONE', *, *, #24449, .T. ) ;
#19353=DIRECTION ( 'NONE',  ( 0.000000000000000000, 0.000000000000000000, 1.000000000000000000 ) ) ;
#19354=CARTESIAN_POINT ( 'NONE',  ( 14.99999999999989342, 2.500000000000000000, -0.7928203230275542301 ) ) ;
#19355=CARTESIAN_POINT ( 'NONE',  ( 12.89999999999990266, 2.500000000000000000, 4.922947341949748257 ) ) ;
#19356=ORIENTED_EDGE ( 'NONE', *, *, #55873, .T. ) ;
#19357=ORIENTED_EDGE ( 'NONE', *, *, #92082, .F. ) ;
#19358=AXIS2_PLACEMENT_3D ( 'NONE', #96535, #27172, #120714 ) ;
#19359=DIRECTION ( 'NONE',  ( 0.000000000000000000, 0.000000000000000000, -1.000000000000000000 ) ) ;
#19360=CARTESIAN_POINT ( 'NONE',  ( -12.09999999999999432, 2.500000000000000000, 3.537306695894645081 ) ) ;
#19362=ORIENTED_EDGE ( 'NONE', *, *, #117460, .F. ) ;
#19363=CARTESIAN_POINT ( 'NONE',  ( 8.349999999999923261, 2.500000000000000000, 2.857883832488649301 ) ) ;
#19364=CIRCLE ( 'NONE', #2638, 0.09999999999999999167 ) ;
#19365=ORIENTED_EDGE ( 'NONE', *, *, #24125, .T. ) ;
#19366=CARTESIAN_POINT ( 'NONE',  ( -2.900000000000030553, 2.500000000000000000, 5.022947341949748790 ) ) ;
#19367=AXIS2_PLACEMENT_3D ( 'NONE', #52013, #42860, #3545 ) ;
#19368=EDGE_CURVE ( 'NONE', #54276, #9000, #46705, .T. ) ;
#19369=COLOUR_RGB ( '', 0.72549020, 0.75294118, 0.79215686) ;
#19370=EDGE_LOOP ( 'NONE', ( #82256, #106139, #122895, #41029 ) ) ;
#19372=DIRECTION ( 'NONE',  ( 0.000000000000000000, 0.000000000000000000, 1.000000000000000000 ) ) ;
#19373=CARTESIAN_POINT ( 'NONE',  ( -7.900000000000011013, 2.500000000000000000, 3.637306695894644726 ) ) ;
#19374=ADVANCED_FACE ( 'NONE', ( #104334 ), #19699, .T. ) ;
#19375=DIRECTION ( 'NONE',  ( 0.000000000000000000, -0.000000000000000000, 1.000000000000000000 ) ) ;
#19376=VECTOR ( 'NONE', #94305, 1000.000000000000000 ) ;
#19377=ADVANCED_FACE ( 'NONE', ( #86620 ), #103701, .T. ) ;
#19378=VERTEX_POINT ( 'NONE', #16574 ) ;
#19379=DIRECTION ( 'NONE',  ( 0.000000000000000000, 1.000000000000000000, 0.000000000000000000 ) ) ;
#19380=AXIS2_PLACEMENT_3D ( 'NONE', #60499, #38938, #30400 ) ;
#19381=EDGE_CURVE ( 'NONE', #22835, #59380, #4180, .T. ) ;
#19382=ORIENTED_EDGE ( 'NONE', *, *, #118544, .T. ) ;
#19383=EDGE_CURVE ( 'NONE', #117981, #27458, #21752, .T. ) ;
#19384=VERTEX_POINT ( 'NONE', #56514 ) ;
#19385=EDGE_CURVE ( 'NONE', #1350, #77225, #115832, .T. ) ;
#19386=LINE ( 'NONE', #59352, #62533 ) ;
#19387=CARTESIAN_POINT ( 'NONE',  ( 0.1999999999999562961, 12.50000000000000000, 4.741630453620009789 ) ) ;
#19388=LINE ( 'NONE', #50172, #111783 ) ;
#19389=EDGE_CURVE ( 'NONE', #34614, #15166, #114787, .T. ) ;
#19391=AXIS2_PLACEMENT_3D ( 'NONE', #17675, #126355, #77881 ) ;
#19392=DIRECTION ( 'NONE',  ( -0.000000000000000000, 1.000000000000000000, -0.000000000000000000 ) ) ;
#19393=DIRECTION ( 'NONE',  ( 0.000000000000000000, 1.000000000000000000, 0.000000000000000000 ) ) ;
#19394=AXIS2_PLACEMENT_3D ( 'NONE', #115901, #47178, #26888 ) ;
#19395=DIRECTION ( 'NONE',  ( -0.000000000000000000, -1.000000000000000000, -0.000000000000000000 ) ) ;
#19396=DIRECTION ( 'NONE',  ( 0.000000000000000000, -0.000000000000000000, 1.000000000000000000 ) ) ;
#19397=AXIS2_PLACEMENT_3D ( 'NONE', #121448, #79137, #19552 ) ;
#19398=VECTOR ( 'NONE', #18384, 1000.000000000000000 ) ;
#19399=DIRECTION ( 'NONE',  ( 0.000000000000000000, -0.9999939076577903929, 0.003490651415223739937 ) ) ;
#19400=EDGE_CURVE ( 'NONE', #114757, #57762, #24488, .T. ) ;
#19402=CONICAL_SURFACE ( 'NONE', #11083, 0.1000000000000002554, 0.003490658503988666988 ) ;
#19405=CARTESIAN_POINT ( 'NONE',  ( 7.299999999999927880, 12.50000000000000000, 4.048810130592458201 ) ) ;
#19406=DIRECTION ( 'NONE',  ( 0.000000000000000000, -0.9999939076577903929, 0.003490651415223739937 ) ) ;
#19407=CARTESIAN_POINT ( 'NONE',  ( 9.149999999999916866, 2.500000000000000000, 7.188010851410848723 ) ) ;
#19408=DIRECTION ( 'NONE',  ( 0.000000000000000000, 0.000000000000000000, 1.000000000000000000 ) ) ;
#19409=VERTEX_POINT ( 'NONE', #14641 ) ;
#19410=DIRECTION ( 'NONE',  ( 0.000000000000000000, 1.000000000000000000, 0.000000000000000000 ) ) ;
#19411=CARTESIAN_POINT ( 'NONE',  ( 7.049999999999926992, 12.50000000000000000, 2.165063509461097713 ) ) ;
#19412=DIRECTION ( 'NONE',  ( 0.000000000000000000, 0.000000000000000000, -1.000000000000000000 ) ) ;
#19413=EDGE_LOOP ( 'NONE', ( #85917, #84895 ) ) ;
#19414=CONICAL_SURFACE ( 'NONE', #92597, 0.09999999999999982514, 0.003490658503988666988 ) ;
#19415=AXIS2_PLACEMENT_3D ( 'NONE', #64810, #33442, #3318 ) ;
#19416=ADVANCED_FACE ( 'NONE', ( #54572 ), #64404, .T. ) ;
#19417=VERTEX_POINT ( 'NONE', #53950 ) ;
#19418=CARTESIAN_POINT ( 'NONE',  ( -5.200000000000025935, 12.50000000000000000, -4.048810130592463530 ) ) ;
#19419=AXIS2_PLACEMENT_3D ( 'NONE', #64669, #65957, #85598 ) ;
#19420=ORIENTED_EDGE ( 'NONE', *, *, #42036, .T. ) ;
#19421=EDGE_LOOP ( 'NONE', ( #25905, #22781 ) ) ;
#19422=VECTOR ( 'NONE', #51058, 1000.000000000000000 ) ;
#19423=ORIENTED_EDGE ( 'NONE', *, *, #2357, .F. ) ;
#19424=LINE ( 'NONE', #78379, #109317 ) ;
#19425=AXIS2_PLACEMENT_3D ( 'NONE', #70550, #43063, #2441 ) ;
#19426=AXIS2_PLACEMENT_3D ( 'NONE', #4897, #36964, #65105 ) ;
#19427=EDGE_CURVE ( 'NONE', #53009, #39225, #93872, .T. ) ;
#19428=CARTESIAN_POINT ( 'NONE',  ( 1.449999999999952660, 2.500000000000000000, -6.741600689897078169 ) ) ;
#19429=DIRECTION ( 'NONE',  ( -0.000000000000000000, 1.000000000000000000, -0.000000000000000000 ) ) ;
#19430=ADVANCED_FACE ( 'NONE', ( #124622 ), #11271, .T. ) ;
#19431=DIRECTION ( 'NONE',  ( 0.000000000000000000, 1.000000000000000000, 0.000000000000000000 ) ) ;
#19433=ORIENTED_EDGE ( 'NONE', *, *, #84749, .T. ) ;
#19434=AXIS2_PLACEMENT_3D ( 'NONE', #69156, #10254, #50198 ) ;
#19435=EDGE_CURVE ( 'NONE', #98451, #88829, #125264, .T. ) ;
#19436=CIRCLE ( 'NONE', #96701, 0.06509327318403745899 ) ;
#19437=DIRECTION ( 'NONE',  ( 0.000000000000000000, 0.000000000000000000, 1.000000000000000000 ) ) ;
#19438=CIRCLE ( 'NONE', #75883, 0.06509327318403745899 ) ;
#19439=ORIENTED_EDGE ( 'NONE', *, *, #19711, .F. ) ;
#19440=PLANE ( 'NONE',  #9894 ) ;
#19441=CONICAL_SURFACE ( 'NONE', #46533, 0.09999999999999982514, 0.003490658503988666988 ) ;
#19442=DIRECTION ( 'NONE',  ( 0.000000000000000000, 0.000000000000000000, 1.000000000000000000 ) ) ;
#19443=DIRECTION ( 'NONE',  ( 0.000000000000000000, 1.000000000000000000, 0.000000000000000000 ) ) ;
#19444=EDGE_CURVE ( 'NONE', #30572, #40528, #5006, .T. ) ;
#19445=FACE_OUTER_BOUND ( 'NONE', #116202, .T. ) ;
#19446=AXIS2_PLACEMENT_3D ( 'NONE', #100859, #19066, #110054 ) ;
#19447=EDGE_CURVE ( 'NONE', #117733, #1262, #15285, .T. ) ;
#19448=ORIENTED_EDGE ( 'NONE', *, *, #13068, .F. ) ;
#19449=EDGE_CURVE ( 'NONE', #69211, #30852, #55244, .T. ) ;
#19450=EDGE_CURVE ( 'NONE', #127530, #96634, #117880, .T. ) ;
#19451=EDGE_LOOP ( 'NONE', ( #13786, #59411, #38414, #79764 ) ) ;
#19452=ORIENTED_EDGE ( 'NONE', *, *, #25619, .T. ) ;
#19453=EDGE_LOOP ( 'NONE', ( #6844, #92308 ) ) ;
#19454=ORIENTED_EDGE ( 'NONE', *, *, #47959, .T. ) ;
#19455=DIRECTION ( 'NONE',  ( 0.000000000000000000, 1.000000000000000000, 0.000000000000000000 ) ) ;
#19456=CARTESIAN_POINT ( 'NONE',  ( -4.150000000000024336, 2.500000000000000000, -2.757883832488654097 ) ) ;
#19457=CARTESIAN_POINT ( 'NONE',  ( -7.900000000000014566, 2.500000000000000000, -3.637306695894650055 ) ) ;
#19458=FACE_BOUND ( 'NONE', #39096, .T. ) ;
#19459=CARTESIAN_POINT ( 'NONE',  ( 0.5999999999999551248, 12.50000000000000000, -4.676537180435978769 ) ) ;
#19460=PLANE ( 'NONE',  #81886 ) ;
#19461=EDGE_CURVE ( 'NONE', #100426, #103079, #122106, .T. ) ;
#19462=DIRECTION ( 'NONE',  ( -0.000000000000000000, 1.000000000000000000, -0.000000000000000000 ) ) ;
#19463=FACE_OUTER_BOUND ( 'NONE', #57604, .T. ) ;
#19464=DIRECTION ( 'NONE',  ( -0.000000000000000000, 1.000000000000000000, -0.000000000000000000 ) ) ;
#19465=CARTESIAN_POINT ( 'NONE',  ( -9.350000000000004974, 2.500000000000000000, 6.841600689897072485 ) ) ;
#19466=FACE_OUTER_BOUND ( 'NONE', #25061, .T. ) ;
#19467=AXIS2_PLACEMENT_3D ( 'NONE', #39904, #81729, #62756 ) ;
#19468=AXIS2_PLACEMENT_3D ( 'NONE', #38838, #118000, #87882 ) ;
#19469=CARTESIAN_POINT ( 'NONE',  ( 7.899999999999923084, 2.500000000000000000, -0.7928203230275543412 ) ) ;
#19470=ORIENTED_EDGE ( 'NONE', *, *, #65269, .T. ) ;
#19471=ORIENTED_EDGE ( 'NONE', *, *, #19557, .T. ) ;
#19472=ORIENTED_EDGE ( 'NONE', *, *, #81741, .F. ) ;
#19473=EDGE_LOOP ( 'NONE', ( #80709, #41385, #88456, #76562 ) ) ;
#19474=DIRECTION ( 'NONE',  ( 0.000000000000000000, 0.000000000000000000, 1.000000000000000000 ) ) ;
#19475=DIRECTION ( 'NONE',  ( -4.274815082592931898E-19, -0.9999939076577903929, -0.003490651415223739937 ) ) ;
#19476=FACE_BOUND ( 'NONE', #53766, .T. ) ;
#19477=CIRCLE ( 'NONE', #34164, 0.1000000000000002554 ) ;
#19478=VECTOR ( 'NONE', #23405, 1000.000000000000000 ) ;
#19479=FACE_OUTER_BOUND ( 'NONE', #363, .T. ) ;
#19480=AXIS2_PLACEMENT_3D ( 'NONE', #119161, #80538, #98871 ) ;
#19481=VECTOR ( 'NONE', #119887, 1000.000000000000000 ) ;
#19482=ORIENTED_EDGE ( 'NONE', *, *, #50915, .T. ) ;
#19483=DIRECTION ( 'NONE',  ( -0.000000000000000000, -1.000000000000000000, -0.000000000000000000 ) ) ;
#19484=DIRECTION ( 'NONE',  ( 0.000000000000000000, 0.000000000000000000, -1.000000000000000000 ) ) ;
#19485=DIRECTION ( 'NONE',  ( 0.000000000000000000, 0.000000000000000000, 1.000000000000000000 ) ) ;
#19486=DIRECTION ( 'NONE',  ( 0.000000000000000000, 0.000000000000000000, 1.000000000000000000 ) ) ;
#19487=DIRECTION ( 'NONE',  ( 0.000000000000000000, 0.000000000000000000, 1.000000000000000000 ) ) ;
#19488=ORIENTED_EDGE ( 'NONE', *, *, #64158, .F. ) ;
#19489=AXIS2_PLACEMENT_3D ( 'NONE', #40418, #48286, #28000 ) ;
#19490=DIRECTION ( 'NONE',  ( 0.000000000000000000, 0.000000000000000000, 1.000000000000000000 ) ) ;
#19491=EDGE_CURVE ( 'NONE', #124192, #17292, #107427, .T. ) ;
#19492=AXIS2_PLACEMENT_3D ( 'NONE', #51990, #111542, #101078 ) ;
#19493=AXIS2_PLACEMENT_3D ( 'NONE', #66400, #25842, #56570 ) ;
#19494=CONICAL_SURFACE ( 'NONE', #67505, 0.1000000000000002554, 0.003490658503988666988 ) ;
#19495=ORIENTED_EDGE ( 'NONE', *, *, #88891, .T. ) ;
#19496=ORIENTED_EDGE ( 'NONE', *, *, #119756, .T. ) ;
#19497=DIRECTION ( 'NONE',  ( -0.000000000000000000, -1.000000000000000000, -0.000000000000000000 ) ) ;
#19498=DIRECTION ( 'NONE',  ( 0.000000000000000000, -0.9999939076577903929, 0.003490651415223739937 ) ) ;
#19499=AXIS2_PLACEMENT_3D ( 'NONE', #10922, #41085, #123471 ) ;
#19500=VERTEX_POINT ( 'NONE', #87258 ) ;
#19501=FACE_OUTER_BOUND ( 'NONE', #19413, .T. ) ;
#19502=DIRECTION ( 'NONE',  ( 0.000000000000000000, 0.000000000000000000, 1.000000000000000000 ) ) ;
#19503=ORIENTED_EDGE ( 'NONE', *, *, #108097, .T. ) ;
#19504=DIRECTION ( 'NONE',  ( 0.000000000000000000, 0.000000000000000000, -1.000000000000000000 ) ) ;
#19506=EDGE_CURVE ( 'NONE', #112250, #40839, #47354, .T. ) ;
#19507=CARTESIAN_POINT ( 'NONE',  ( -9.350000000000008527, 2.500000000000000000, -6.148780366869520897 ) ) ;
#19508=EDGE_LOOP ( 'NONE', ( #58858, #90991, #115167, #97260 ) ) ;
#19509=CARTESIAN_POINT ( 'NONE',  ( -0.2000000000000404232, 2.500000000000000000, 4.083716857408421497 ) ) ;
#19510=FACE_BOUND ( 'NONE', #119146, .T. ) ;
#19511=EDGE_LOOP ( 'NONE', ( #51870, #72439 ) ) ;
#19512=CARTESIAN_POINT ( 'NONE',  ( 5.399999999999933742, 2.500000000000000000, 0.09999999999999761857 ) ) ;
#19513=ORIENTED_EDGE ( 'NONE', *, *, #58525, .F. ) ;
#19515=CARTESIAN_POINT ( 'NONE',  ( -10.80000000000000249, 2.500000000000000000, -4.330127018922197202 ) ) ;
#19516=CIRCLE ( 'NONE', #21577, 0.06509327318403745899 ) ;
#19517=CARTESIAN_POINT ( 'NONE',  ( 4.199999999999938005, 2.500000000000000000, 4.330127018922196314 ) ) ;
#19518=AXIS2_PLACEMENT_3D ( 'NONE', #111238, #22897, #41895 ) ;
#19521=VERTEX_POINT ( 'NONE', #68913 ) ;
#19523=ORIENTED_EDGE ( 'NONE', *, *, #66114, .F. ) ;
#19524=DIRECTION ( 'NONE',  ( 0.000000000000000000, 0.000000000000000000, 1.000000000000000000 ) ) ;
#19525=CIRCLE ( 'NONE', #119879, 0.06509327318403745899 ) ;
#19526=CIRCLE ( 'NONE', #76062, 0.06509327318403741736 ) ;
#19527=DIRECTION ( 'NONE',  ( -0.000000000000000000, -1.000000000000000000, -0.000000000000000000 ) ) ;
#19528=AXIS2_PLACEMENT_3D ( 'NONE', #4361, #84229, #126758 ) ;
#19529=CARTESIAN_POINT ( 'NONE',  ( 1.049999999999952971, 2.500000000000000000, 6.248780366869521430 ) ) ;
#19530=EDGE_LOOP ( 'NONE', ( #46823, #81014 ) ) ;
#19531=ORIENTED_EDGE ( 'NONE', *, *, #73398, .F. ) ;
#19532=EDGE_LOOP ( 'NONE', ( #59531, #123960 ) ) ;
#19533=CARTESIAN_POINT ( 'NONE',  ( 97.50000000000000000, 2.449293598294706414E-16, -2.000000000000000000 ) ) ;
#19534=CARTESIAN_POINT ( 'NONE',  ( 11.89999999999990798, 2.500000000000000000, 4.676537180435972552 ) ) ;
#19535=AXIS2_PLACEMENT_3D ( 'NONE', #38617, #109255, #29427 ) ;
#19536=VECTOR ( 'NONE', #19180, 1000.000000000000000 ) ;
#19537=AXIS2_PLACEMENT_3D ( 'NONE', #2902, #43481, #42856 ) ;
#19538=EDGE_CURVE ( 'NONE', #86078, #28471, #128384, .T. ) ;
#19540=CARTESIAN_POINT ( 'NONE',  ( 1.899999999999951283, 2.500000000000000000, 0.3464101615137736845 ) ) ;
#19541=CARTESIAN_POINT ( 'NONE',  ( -2.100000000000033840, 2.500000000000000000, 3.537306695894645081 ) ) ;
#19542=FACE_OUTER_BOUND ( 'NONE', #74126, .T. ) ;
#19543=CIRCLE ( 'NONE', #126151, 0.06509327318403745899 ) ;
#19544=CARTESIAN_POINT ( 'NONE',  ( 2.899999999999943956, 2.500000000000000000, 4.230127018922196669 ) ) ;
#19546=DIRECTION ( 'NONE',  ( 0.000000000000000000, 1.000000000000000000, 0.000000000000000000 ) ) ;
#19547=AXIS2_PLACEMENT_3D ( 'NONE', #121788, #62887, #112635 ) ;
#19548=EDGE_CURVE ( 'NONE', #94029, #30530, #80249, .T. ) ;
#19549=ORIENTED_EDGE ( 'NONE', *, *, #104637, .T. ) ;
#19550=ORIENTED_EDGE ( 'NONE', *, *, #38222, .T. ) ;
#19551=CARTESIAN_POINT ( 'NONE',  ( 9.149999999999920419, 2.500000000000000000, 2.857883832488649301 ) ) ;
#19552=DIRECTION ( 'NONE',  ( 0.000000000000000000, 0.000000000000000000, 1.000000000000000000 ) ) ;
#19553=EDGE_CURVE ( 'NONE', #123660, #106056, #86491, .T. ) ;
#19554=ORIENTED_EDGE ( 'NONE', *, *, #24859, .T. ) ;
#19555=EDGE_CURVE ( 'NONE', #93259, #41595, #124146, .T. ) ;
#19556=EDGE_LOOP ( 'NONE', ( #46189, #40892 ) ) ;
#19557=EDGE_CURVE ( 'NONE', #106765, #66380, #84445, .T. ) ;
#19559=DIRECTION ( 'NONE',  ( -0.000000000000000000, 1.000000000000000000, -0.000000000000000000 ) ) ;
#19560=ADVANCED_FACE ( 'NONE', ( #9358 ), #28009, .T. ) ;
#19561=ADVANCED_FACE ( 'NONE', ( #28361 ), #71937, .T. ) ;
#19562=CARTESIAN_POINT ( 'NONE',  ( 2.500000000000002220, 1.500000000000000444, -9.999999999999998224 ) ) ;
#19563=CONICAL_SURFACE ( 'NONE', #92726, 0.1000000000000000472, 0.003490658503988666988 ) ;
#19564=CARTESIAN_POINT ( 'NONE',  ( -2.050000000000032685, 2.500000000000000000, -2.165063509461101710 ) ) ;
#19565=DIRECTION ( 'NONE',  ( 0.000000000000000000, 0.000000000000000000, 1.000000000000000000 ) ) ;
#19566=CARTESIAN_POINT ( 'NONE',  ( 2.499999999999948930, 2.500000000000000000, -5.122947341949753763 ) ) ;
#19567=DIRECTION ( 'NONE',  ( -0.000000000000000000, 1.000000000000000000, -0.000000000000000000 ) ) ;
#19568=EDGE_CURVE ( 'NONE', #101562, #116228, #69870, .T. ) ;
#19569=CIRCLE ( 'NONE', #94781, 0.1000000000000002554 ) ;
#19571=CIRCLE ( 'NONE', #92734, 0.1000000000000002554 ) ;
#19572=EDGE_CURVE ( 'NONE', #70666, #69440, #99121, .T. ) ;
#19574=ADVANCED_FACE ( 'NONE', ( #87893 ), #127839, .T. ) ;
#19575=ORIENTED_EDGE ( 'NONE', *, *, #71733, .F. ) ;
#19576=ORIENTED_EDGE ( 'NONE', *, *, #114404, .F. ) ;
#19577=ORIENTED_EDGE ( 'NONE', *, *, #98575, .T. ) ;
#19578=VERTEX_POINT ( 'NONE', #89202 ) ;
#19579=VECTOR ( 'NONE', #36558, 1000.000000000000000 ) ;
#19580=CARTESIAN_POINT ( 'NONE',  ( 1.699999999999950218, 2.500000000000000000, 4.230127018922196669 ) ) ;
#19581=DIRECTION ( 'NONE',  ( 0.000000000000000000, 0.000000000000000000, -1.000000000000000000 ) ) ;
#19582=AXIS2_PLACEMENT_3D ( 'NONE', #63841, #105033, #113584 ) ;
#19583=CONICAL_SURFACE ( 'NONE', #36224, 0.09999999999999982514, 0.003490658503988666988 ) ;
#19584=ORIENTED_EDGE ( 'NONE', *, *, #28109, .T. ) ;
#19585=DIRECTION ( 'NONE',  ( -4.274815082592931898E-19, -0.9999939076577903929, -0.003490651415223739937 ) ) ;
#19586=CIRCLE ( 'NONE', #78069, 0.06509327318403745899 ) ;
#19587=CARTESIAN_POINT ( 'NONE',  ( 4.799999999999935874, 2.500000000000000000, 4.083716857408421497 ) ) ;
#19588=CARTESIAN_POINT ( 'NONE',  ( 2.099999999999950351, 12.50000000000000000, -5.088040615133791356 ) ) ;
#19589=DIRECTION ( 'NONE',  ( 0.000000000000000000, 1.000000000000000000, 0.000000000000000000 ) ) ;
#19590=EDGE_LOOP ( 'NONE', ( #126768, #95847, #41194, #17640 ) ) ;
#19591=DIRECTION ( 'NONE',  ( 0.000000000000000000, 0.000000000000000000, 1.000000000000000000 ) ) ;
#19592=CIRCLE ( 'NONE', #13312, 0.09999999999999982514 ) ;
#19593=DIRECTION ( 'NONE',  ( -0.000000000000000000, 1.000000000000000000, -0.000000000000000000 ) ) ;
#19594=ORIENTED_EDGE ( 'NONE', *, *, #118546, .F. ) ;
#19595=AXIS2_PLACEMENT_3D ( 'NONE', #119263, #40075, #19113 ) ;
#19596=AXIS2_PLACEMENT_3D ( 'NONE', #651, #57655, #28193 ) ;
#19597=AXIS2_PLACEMENT_3D ( 'NONE', #59325, #99232, #27247 ) ;
#19598=EDGE_LOOP ( 'NONE', ( #55170, #63083 ) ) ;
#19599=EDGE_LOOP ( 'NONE', ( #45999, #37101, #75251, #58764 ) ) ;
#19600=VERTEX_POINT ( 'NONE', #78104 ) ;
#19601=CARTESIAN_POINT ( 'NONE',  ( -2.700000000000030376, 12.50000000000000000, 3.983716857408420964 ) ) ;
#19602=AXIS2_PLACEMENT_3D ( 'NONE', #12081, #60569, #72311 ) ;
#19604=LINE ( 'NONE', #69326, #73239 ) ;
#19605=AXIS2_PLACEMENT_3D ( 'NONE', #18507, #127815, #17857 ) ;
#19606=ORIENTED_EDGE ( 'NONE', *, *, #71310, .T. ) ;
#19607=CARTESIAN_POINT ( 'NONE',  ( -9.600000000000008527, 2.500000000000000000, 4.430127018922196847 ) ) ;
#19608=DIRECTION ( 'NONE',  ( 0.000000000000000000, 0.000000000000000000, -1.000000000000000000 ) ) ;
#19609=CARTESIAN_POINT ( 'NONE',  ( -10.65000000000000213, 2.500000000000000000, 6.248780366869520542 ) ) ;
#19611=EDGE_CURVE ( 'NONE', #98546, #52824, #7056, .T. ) ;
#19612=ADVANCED_FACE ( 'NONE', ( #18526 ), #53145, .T. ) ;
#19613=ORIENTED_EDGE ( 'NONE', *, *, #53378, .F. ) ;
#19615=EDGE_CURVE ( 'NONE', #77606, #64779, #8685, .T. ) ;
#19616=EDGE_LOOP ( 'NONE', ( #94872, #78363, #95697, #59410 ) ) ;
#19617=EDGE_LOOP ( 'NONE', ( #38079, #2624 ) ) ;
#19618=FACE_OUTER_BOUND ( 'NONE', #48682, .T. ) ;
#19619=AXIS2_PLACEMENT_3D ( 'NONE', #34548, #124842, #16143 ) ;
#19620=CIRCLE ( 'NONE', #117791, 0.1000000000000002554 ) ;
#19621=CARTESIAN_POINT ( 'NONE',  ( 9.549999999999918998, 2.500000000000000000, -6.595190528383302109 ) ) ;
#19622=FACE_BOUND ( 'NONE', #102299, .T. ) ;
#19623=CARTESIAN_POINT ( 'NONE',  ( 3.749999999999975131, 12.50000000000000000, 6.560283801567334372 ) ) ;
#19625=ADVANCED_FACE ( 'NONE', ( #78762 ), #86576, .T. ) ;
#19626=DIRECTION ( 'NONE',  ( 0.000000000000000000, 0.000000000000000000, 1.000000000000000000 ) ) ;
#19627=CIRCLE ( 'NONE', #7077, 0.1000000000000002554 ) ;
#19628=AXIS2_PLACEMENT_3D ( 'NONE', #116305, #26018, #26659 ) ;
#19630=CONICAL_SURFACE ( 'NONE', #124179, 0.09999999999999999167, 0.003490658503988666988 ) ;
#19631=VECTOR ( 'NONE', #70137, 1000.000000000000000 ) ;
#19632=EDGE_LOOP ( 'NONE', ( #111815, #75720, #61324, #11660 ) ) ;
#19633=FACE_OUTER_BOUND ( 'NONE', #74323, .T. ) ;
#19634=FACE_OUTER_BOUND ( 'NONE', #67407, .T. ) ;
#19636=DIRECTION ( 'NONE',  ( -0.000000000000000000, -1.000000000000000000, -0.000000000000000000 ) ) ;
#19637=ORIENTED_EDGE ( 'NONE', *, *, #52778, .F. ) ;
#19638=CONICAL_SURFACE ( 'NONE', #36375, 0.1000000000000002554, 0.003490658503988666988 ) ;
#19640=AXIS2_PLACEMENT_3D ( 'NONE', #66071, #73969, #85074 ) ;
#19641=AXIS2_PLACEMENT_3D ( 'NONE', #6098, #126545, #25753 ) ;
#19642=DIRECTION ( 'NONE',  ( 0.000000000000000000, 0.000000000000000000, -1.000000000000000000 ) ) ;
#19643=EDGE_LOOP ( 'NONE', ( #98365, #10971, #29002, #129560 ) ) ;
#19644=VERTEX_POINT ( 'NONE', #119299 ) ;
#19645=AXIS2_PLACEMENT_3D ( 'NONE', #19731, #11178, #59675 ) ;
#19646=CARTESIAN_POINT ( 'NONE',  ( 4.549999999999935874, 12.50000000000000000, 6.495190528383297135 ) ) ;
#19647=DIRECTION ( 'NONE',  ( 0.000000000000000000, 1.000000000000000000, 0.000000000000000000 ) ) ;
#19648=EDGE_CURVE ( 'NONE', #40995, #64274, #17527, .T. ) ;
#19649=FACE_BOUND ( 'NONE', #14100, .T. ) ;
#19650=CARTESIAN_POINT ( 'NONE',  ( 10.04522989427051982, -2.499999999999999112, -8.164691043833789408 ) ) ;
#19651=CARTESIAN_POINT ( 'NONE',  ( 4.999999999999935163, 2.500000000000000000, 0.6928203230275494784 ) ) ;
#19652=ORIENTED_EDGE ( 'NONE', *, *, #117855, .F. ) ;
#19653=CARTESIAN_POINT ( 'NONE',  ( 9.149999999999920419, 12.50000000000000000, 1.407149913249508000 ) ) ;
#19655=AXIS2_PLACEMENT_3D ( 'NONE', #77887, #29455, #39303 ) ;
#19656=EDGE_LOOP ( 'NONE', ( #14533, #11589 ) ) ;
#19657=DIRECTION ( 'NONE',  ( -0.000000000000000000, -1.000000000000000000, -0.000000000000000000 ) ) ;
#19658=CARTESIAN_POINT ( 'NONE',  ( -8.100000000000013856, 12.50000000000000000, -4.676537180435977881 ) ) ;
#19659=EDGE_CURVE ( 'NONE', #77218, #115634, #111636, .T. ) ;
#19660=DIRECTION ( 'NONE',  ( 0.000000000000000000, 1.000000000000000000, 0.000000000000000000 ) ) ;
#19661=DIRECTION ( 'NONE',  ( 0.000000000000000000, 0.000000000000000000, 1.000000000000000000 ) ) ;
#19662=CONICAL_SURFACE ( 'NONE', #111696, 0.1000000000000002554, 0.003490658503988666988 ) ;
#19663=AXIS2_PLACEMENT_3D ( 'NONE', #115213, #28164, #37349 ) ;
#19664=ORIENTED_EDGE ( 'NONE', *, *, #45144, .F. ) ;
#19665=CARTESIAN_POINT ( 'NONE',  ( -7.900000000000014566, 2.500000000000000000, 0.6928203230275494784 ) ) ;
#19666=DIRECTION ( 'NONE',  ( -0.000000000000000000, -1.000000000000000000, -0.000000000000000000 ) ) ;
#19667=CARTESIAN_POINT ( 'NONE',  ( 8.349999999999923261, 2.500000000000000000, -6.495190528383302464 ) ) ;
#19668=DIRECTION ( 'NONE',  ( -0.000000000000000000, -1.000000000000000000, -0.000000000000000000 ) ) ;
#19669=VERTEX_POINT ( 'NONE', #97093 ) ;
#19671=EDGE_CURVE ( 'NONE', #42458, #40528, #110765, .T. ) ;
#19672=AXIS2_PLACEMENT_3D ( 'NONE', #127502, #60066, #79678 ) ;
#19673=CARTESIAN_POINT ( 'NONE',  ( 6.699999999999930012, 12.50000000000000000, 4.330127018922196314 ) ) ;
#19674=ORIENTED_EDGE ( 'NONE', *, *, #104362, .F. ) ;
#19675=CIRCLE ( 'NONE', #40535, 0.1000000000000002554 ) ;
#19676=DIRECTION ( 'NONE',  ( 0.000000000000000000, 0.000000000000000000, -1.000000000000000000 ) ) ;
#19677=DIRECTION ( 'NONE',  ( 0.000000000000000000, 0.000000000000000000, -1.000000000000000000 ) ) ;
#19678=AXIS2_PLACEMENT_3D ( 'NONE', #129423, #111011, #111690 ) ;
#19679=CARTESIAN_POINT ( 'NONE',  ( -1.250000000000037526, 12.50000000000000000, -1.472243186433550122 ) ) ;
#19680=ORIENTED_EDGE ( 'NONE', *, *, #111436, .T. ) ;
#19682=CARTESIAN_POINT ( 'NONE',  ( 8.749999999999918288, 2.500000000000000000, -1.472243186433550122 ) ) ;
#19683=CARTESIAN_POINT ( 'NONE',  ( 12.09999999999990550, 12.50000000000000000, 4.330127018922196314 ) ) ;
#19684=EDGE_CURVE ( 'NONE', #85856, #55123, #92956, .T. ) ;
#19685=FACE_OUTER_BOUND ( 'NONE', #78952, .T. ) ;
#19686=CARTESIAN_POINT ( 'NONE',  ( 1.649999999999951505, 12.50000000000000000, 1.472243186433545459 ) ) ;
#19687=DIRECTION ( 'NONE',  ( 0.000000000000000000, 1.000000000000000000, 0.000000000000000000 ) ) ;
#19688=ORIENTED_EDGE ( 'NONE', *, *, #4010, .T. ) ;
#19689=ORIENTED_EDGE ( 'NONE', *, *, #100437, .T. ) ;
#19690=DIRECTION ( 'NONE',  ( 0.000000000000000000, -0.000000000000000000, 1.000000000000000000 ) ) ;
#19691=VECTOR ( 'NONE', #25566, 1000.000000000000000 ) ;
#19692=ORIENTED_EDGE ( 'NONE', *, *, #115021, .T. ) ;
#19693=AXIS2_PLACEMENT_3D ( 'NONE', #99934, #29896, #129419 ) ;
#19694=CIRCLE ( 'NONE', #90700, 0.06509327318403743123 ) ;
#19695=DIRECTION ( 'NONE',  ( -0.000000000000000000, -1.000000000000000000, -0.000000000000000000 ) ) ;
#19696=ORIENTED_EDGE ( 'NONE', *, *, #4625, .F. ) ;
#19697=ORIENTED_EDGE ( 'NONE', *, *, #127276, .F. ) ;
#19698=ORIENTED_EDGE ( 'NONE', *, *, #41322, .T. ) ;
#19699=CONICAL_SURFACE ( 'NONE', #9230, 0.09999999999999982514, 0.003490658503988666988 ) ;
#19700=CARTESIAN_POINT ( 'NONE',  ( 13.34999999999990017, 12.50000000000000000, 2.165063509461097713 ) ) ;
#19701=CARTESIAN_POINT ( 'NONE',  ( -10.60000000000000142, 2.500000000000000000, 0.3464101615137736845 ) ) ;
#19702=CARTESIAN_POINT ( 'NONE',  ( 6.849999999999930367, 2.500000000000000000, -6.148780366869526226 ) ) ;
#19703=EDGE_CURVE ( 'NONE', #58714, #48991, #38590, .T. ) ;
#19704=DIRECTION ( 'NONE',  ( -0.000000000000000000, -1.000000000000000000, -0.000000000000000000 ) ) ;
#19705=CARTESIAN_POINT ( 'NONE',  ( -14.79999999999998472, 2.500000000000000000, 0.4464101615137758272 ) ) ;
#19707=DIRECTION ( 'NONE',  ( -0.000000000000000000, -1.000000000000000000, -0.000000000000000000 ) ) ;
#19708=DIRECTION ( 'NONE',  ( -0.000000000000000000, -1.000000000000000000, -0.000000000000000000 ) ) ;
#19709=FACE_OUTER_BOUND ( 'NONE', #127559, .T. ) ;
#19710=ORIENTED_EDGE ( 'NONE', *, *, #111809, .T. ) ;
#19711=EDGE_CURVE ( 'NONE', #89250, #47871, #86675, .T. ) ;
#19712=ORIENTED_EDGE ( 'NONE', *, *, #83699, .F. ) ;
#19713=CONICAL_SURFACE ( 'NONE', #111736, 0.1000000000000002554, 0.003490658503988666988 ) ;
#19714=FACE_OUTER_BOUND ( 'NONE', #88999, .T. ) ;
#19715=AXIS2_PLACEMENT_3D ( 'NONE', #37750, #88101, #49515 ) ;
#19716=EDGE_CURVE ( 'NONE', #73117, #89300, #97051, .T. ) ;
#19717=AXIS2_PLACEMENT_3D ( 'NONE', #100628, #10332, #10945 ) ;
#19718=ORIENTED_EDGE ( 'NONE', *, *, #31540, .T. ) ;
#19719=EDGE_CURVE ( 'NONE', #74320, #86613, #55292, .T. ) ;
#19720=ORIENTED_EDGE ( 'NONE', *, *, #1118, .F. ) ;
#19721=EDGE_CURVE ( 'NONE', #125242, #7618, #122537, .T. ) ;
#19722=CARTESIAN_POINT ( 'NONE',  ( 11.64999999999990798, 2.500000000000000000, -1.472243186433550122 ) ) ;
#19723=ADVANCED_FACE ( 'NONE', ( #100944 ), #7154, .T. ) ;
#19724=CIRCLE ( 'NONE', #92891, 0.06509327318403745899 ) ;
#19725=AXIS2_PLACEMENT_3D ( 'NONE', #31186, #39729, #50180 ) ;
#19726=DIRECTION ( 'NONE',  ( -0.000000000000000000, 1.000000000000000000, -0.000000000000000000 ) ) ;
#19727=CIRCLE ( 'NONE', #122224, 0.1000000000000002554 ) ;
#19728=DIRECTION ( 'NONE',  ( -0.000000000000000000, -1.000000000000000000, -0.000000000000000000 ) ) ;
#19729=CARTESIAN_POINT ( 'NONE',  ( -4.550000000000022915, 2.500000000000000000, 6.495190528383297135 ) ) ;
#19730=EDGE_CURVE ( 'NONE', #125465, #13400, #26046, .T. ) ;
#19731=CARTESIAN_POINT ( 'NONE',  ( 13.09999999999990195, 12.50000000000000000, 4.676537180435972552 ) ) ;
#19732=EDGE_LOOP ( 'NONE', ( #45833, #83758 ) ) ;
#19733=EDGE_CURVE ( 'NONE', #48204, #86305, #32333, .T. ) ;
#19734=ADVANCED_FACE ( 'NONE', ( #70856 ), #81326, .T. ) ;
#19735=VECTOR ( 'NONE', #21371, 1000.000000000000000 ) ;
#19736=ADVANCED_FACE ( 'NONE', ( #60412 ), #36525, .T. ) ;
#19737=ORIENTED_EDGE ( 'NONE', *, *, #69680, .F. ) ;
#19738=DIRECTION ( 'NONE',  ( -0.000000000000000000, -1.000000000000000000, -0.000000000000000000 ) ) ;
#19739=CIRCLE ( 'NONE', #115863, 0.09999999999999982514 ) ;
#19740=ADVANCED_FACE ( 'NONE', ( #112719 ), #120598, .T. ) ;
#19741=VERTEX_POINT ( 'NONE', #23045 ) ;
#19742=CARTESIAN_POINT ( 'NONE',  ( 13.09999999999989839, 2.500000000000000000, 0.3464101615137735735 ) ) ;
#19743=ORIENTED_EDGE ( 'NONE', *, *, #10574, .F. ) ;
#19744=VECTOR ( 'NONE', #6481, 1000.000000000000000 ) ;
#19745=ORIENTED_EDGE ( 'NONE', *, *, #96121, .T. ) ;
#19746=ADVANCED_FACE ( 'NONE', ( #112072 ), #62335, .T. ) ;
#19747=PLANE ( 'NONE',  #125526 ) ;
#19748=CARTESIAN_POINT ( 'NONE',  ( 5.199999999999933564, 2.500000000000000000, 0.2464101615137735679 ) ) ;
#19749=CARTESIAN_POINT ( 'NONE',  ( -8.300000000000009592, 12.50000000000000000, 4.330127018922196314 ) ) ;
#19750=DIRECTION ( 'NONE',  ( -4.274815082592931898E-19, -0.9999939076577903929, -0.003490651415223739937 ) ) ;
#19751=DIRECTION ( 'NONE',  ( 0.000000000000000000, 0.000000000000000000, 1.000000000000000000 ) ) ;
#19752=ORIENTED_EDGE ( 'NONE', *, *, #70959, .T. ) ;
#19753=DIRECTION ( 'NONE',  ( 0.000000000000000000, 0.000000000000000000, -1.000000000000000000 ) ) ;
#19754=CARTESIAN_POINT ( 'NONE',  ( 8.149999999999923972, 2.500000000000000000, -6.841600689897077814 ) ) ;
#19755=DIRECTION ( 'NONE',  ( 0.000000000000000000, 0.000000000000000000, 1.000000000000000000 ) ) ;
#19756=CARTESIAN_POINT ( 'NONE',  ( 14.39999999999989555, 12.50000000000000000, -0.3464101615137782364 ) ) ;
#19757=FACE_OUTER_BOUND ( 'NONE', #10532, .T. ) ;
#19758=VERTEX_POINT ( 'NONE', #62964 ) ;
#19759=VERTEX_POINT ( 'NONE', #52493 ) ;
#19760=CARTESIAN_POINT ( 'NONE',  ( -10.40000000000000213, 2.500000000000000000, -4.430127018922197735 ) ) ;
#19761=ORIENTED_EDGE ( 'NONE', *, *, #103584, .F. ) ;
#19762=AXIS2_PLACEMENT_3D ( 'NONE', #126721, #76973, #67112 ) ;
#19763=CARTESIAN_POINT ( 'NONE',  ( 13.34999999999989662, 2.500000000000000000, -2.957883832488653830 ) ) ;
#19764=CARTESIAN_POINT ( 'NONE',  ( -13.14999999999999147, 12.50000000000000000, 2.446380397790839822 ) ) ;
#19765=VECTOR ( 'NONE', #112536, 1000.000000000000000 ) ;
#19766=EDGE_LOOP ( 'NONE', ( #113661, #2123, #18677, #32329 ) ) ;
#19767=FACE_OUTER_BOUND ( 'NONE', #83306, .T. ) ;
#19768=DIRECTION ( 'NONE',  ( -0.000000000000000000, 1.000000000000000000, -0.000000000000000000 ) ) ;
#19769=CARTESIAN_POINT ( 'NONE',  ( 8.749999999999918288, 12.50000000000000000, 7.188010851410848723 ) ) ;
#19770=DIRECTION ( 'NONE',  ( 0.000000000000000000, 0.000000000000000000, 1.000000000000000000 ) ) ;
#19771=CONICAL_SURFACE ( 'NONE', #128455, 0.09999999999999982514, 0.003490658503988666988 ) ;
#19772=EDGE_CURVE ( 'NONE', #78977, #98217, #124249, .T. ) ;
#19773=DIRECTION ( 'NONE',  ( 0.000000000000000000, 0.000000000000000000, 1.000000000000000000 ) ) ;
#19774=CIRCLE ( 'NONE', #53232, 0.09999999999999982514 ) ;
#19775=EDGE_CURVE ( 'NONE', #85514, #87169, #63608, .T. ) ;
#19776=ORIENTED_EDGE ( 'NONE', *, *, #11944, .F. ) ;
#19777=DIRECTION ( 'NONE',  ( 0.000000000000000000, 0.000000000000000000, -1.000000000000000000 ) ) ;
#19778=DIRECTION ( 'NONE',  ( -0.000000000000000000, 1.000000000000000000, -0.000000000000000000 ) ) ;
#19779=DIRECTION ( 'NONE',  ( -0.000000000000000000, 1.000000000000000000, -0.000000000000000000 ) ) ;
#19780=EDGE_CURVE ( 'NONE', #83439, #89946, #117967, .T. ) ;
#19781=ORIENTED_EDGE ( 'NONE', *, *, #31835, .F. ) ;
#19782=VECTOR ( 'NONE', #78574, 1000.000000000000000 ) ;
#19784=CARTESIAN_POINT ( 'NONE',  ( 11.64999999999990621, 2.500000000000000000, -2.065063509461102065 ) ) ;
#19785=CONICAL_SURFACE ( 'NONE', #126391, 0.09999999999999982514, 0.003490658503988666988 ) ;
#19786=ORIENTED_EDGE ( 'NONE', *, *, #71988, .F. ) ;
#19787=CARTESIAN_POINT ( 'NONE',  ( -6.650000000000014566, 2.500000000000000000, 1.472243186433545459 ) ) ;
#19788=LINE ( 'NONE', #18485, #6914 ) ;
#19789=DIRECTION ( 'NONE',  ( 0.000000000000000000, 1.000000000000000000, 0.000000000000000000 ) ) ;
#19790=AXIS2_PLACEMENT_3D ( 'NONE', #91919, #71629, #41550 ) ;
#19791=VERTEX_POINT ( 'NONE', #93086 ) ;
#19792=DIRECTION ( 'NONE',  ( 0.000000000000000000, 0.000000000000000000, -1.000000000000000000 ) ) ;
#19793=CARTESIAN_POINT ( 'NONE',  ( -13.09999999999999254, 2.500000000000000000, 0.3464101615137777923 ) ) ;
#19794=ORIENTED_EDGE ( 'NONE', *, *, #104993, .T. ) ;
#19795=CARTESIAN_POINT ( 'NONE',  ( 3.349999999999943689, 2.500000000000000000, 2.065063509461097624 ) ) ;
#19796=VERTEX_POINT ( 'NONE', #3399 ) ;
#19797=CARTESIAN_POINT ( 'NONE',  ( 1.049999999999954081, 2.500000000000000000, -6.248780366869526759 ) ) ;
#19799=ORIENTED_EDGE ( 'NONE', *, *, #79658, .T. ) ;
#19800=DIRECTION ( 'NONE',  ( -0.000000000000000000, 1.000000000000000000, -0.000000000000000000 ) ) ;
#19801=CARTESIAN_POINT ( 'NONE',  ( 9.149999999999916866, 2.500000000000000000, 5.902370205355745192 ) ) ;
#19802=AXIS2_PLACEMENT_3D ( 'NONE', #1053, #77670, #49526 ) ;
#19803=AXIS2_PLACEMENT_3D ( 'NONE', #29079, #78826, #79463 ) ;
#19804=AXIS2_PLACEMENT_3D ( 'NONE', #24031, #65213, #105806 ) ;
#19805=ORIENTED_EDGE ( 'NONE', *, *, #22918, .F. ) ;
#19806=EDGE_LOOP ( 'NONE', ( #97022, #113275 ) ) ;
#19807=DIRECTION ( 'NONE',  ( 0.000000000000000000, -0.000000000000000000, 1.000000000000000000 ) ) ;
#19808=CARTESIAN_POINT ( 'NONE',  ( -6.650000000000018119, 2.500000000000000000, -7.188010851410854052 ) ) ;
#19809=ORIENTED_EDGE ( 'NONE', *, *, #17602, .F. ) ;
#19810=DIRECTION ( 'NONE',  ( 0.000000000000000000, 1.000000000000000000, 0.000000000000000000 ) ) ;
#19811=EDGE_CURVE ( 'NONE', #74459, #115955, #44837, .T. ) ;
#19812=CARTESIAN_POINT ( 'NONE',  ( -9.150000000000009237, 2.500000000000000000, -6.495190528383297135 ) ) ;
#19813=AXIS2_PLACEMENT_3D ( 'NONE', #54167, #31954, #93440 ) ;
#19814=AXIS2_PLACEMENT_3D ( 'NONE', #75845, #115781, #34670 ) ;
#19815=AXIS2_PLACEMENT_3D ( 'NONE', #46768, #4879, #74294 ) ;
#19816=DIRECTION ( 'NONE',  ( 0.000000000000000000, 0.000000000000000000, 1.000000000000000000 ) ) ;
#19817=CARTESIAN_POINT ( 'NONE',  ( -12.29999999999999716, 2.500000000000000000, -3.983716857408423628 ) ) ;
#19818=DIRECTION ( 'NONE',  ( 0.000000000000000000, -0.9999939076577903929, 0.003490651415223739937 ) ) ;
#19819=AXIS2_PLACEMENT_3D ( 'NONE', #50337, #90238, #20879 ) ;
#19820=DIRECTION ( 'NONE',  ( -0.000000000000000000, 1.000000000000000000, -0.000000000000000000 ) ) ;
#19821=CARTESIAN_POINT ( 'NONE',  ( -3.100000000000028511, 2.500000000000000000, -3.983716857408426293 ) ) ;
#19822=VECTOR ( 'NONE', #92012, 1000.000000000000000 ) ;
#19823=ORIENTED_EDGE ( 'NONE', *, *, #3542, .T. ) ;
#19824=VERTEX_POINT ( 'NONE', #43341 ) ;
#19825=ORIENTED_EDGE ( 'NONE', *, *, #25416, .T. ) ;
#19826=ORIENTED_EDGE ( 'NONE', *, *, #76141, .F. ) ;
#19827=DIRECTION ( 'NONE',  ( 0.000000000000000000, 0.000000000000000000, 1.000000000000000000 ) ) ;
#19828=DIRECTION ( 'NONE',  ( 0.000000000000000000, 0.000000000000000000, 1.000000000000000000 ) ) ;
#19829=CIRCLE ( 'NONE', #128518, 0.1000000000000002554 ) ;
#19830=EDGE_CURVE ( 'NONE', #21708, #67757, #49051, .T. ) ;
#19831=CARTESIAN_POINT ( 'NONE',  ( -5.000000000000026645, 2.500000000000000000, -3.637306695894650055 ) ) ;
#19832=ORIENTED_EDGE ( 'NONE', *, *, #110608, .F. ) ;
#19833=FACE_BOUND ( 'NONE', #44160, .T. ) ;
#19834=ORIENTED_EDGE ( 'NONE', *, *, #48232, .F. ) ;
#19835=ADVANCED_FACE ( 'NONE', ( #73419 ), #115927, .T. ) ;
#19836=DIRECTION ( 'NONE',  ( 0.000000000000000000, 1.000000000000000000, 0.000000000000000000 ) ) ;
#19837=DIRECTION ( 'NONE',  ( 0.000000000000000000, 1.000000000000000000, 0.000000000000000000 ) ) ;
#19838=DIRECTION ( 'NONE',  ( 0.000000000000000000, 1.000000000000000000, 0.000000000000000000 ) ) ;
#19839=CARTESIAN_POINT ( 'NONE',  ( 16.56576425165006583, 1.500000000000000888, -6.084390597445814564 ) ) ;
#19840=CARTESIAN_POINT ( 'NONE',  ( -6.650000000000014566, 2.500000000000000000, 1.372243186433545370 ) ) ;
#19841=DIRECTION ( 'NONE',  ( 0.000000000000000000, -0.9999939076577903929, 0.003490651415223739937 ) ) ;
#19842=CARTESIAN_POINT ( 'NONE',  ( 8.549999999999918998, 12.50000000000000000, -1.818653347947326138 ) ) ;
#19843=CARTESIAN_POINT ( 'NONE',  ( -1.700000000000034817, 2.500000000000000000, -2.385244779468109755E-15 ) ) ;
#19844=EDGE_CURVE ( 'NONE', #110912, #113131, #61567, .T. ) ;
#19845=CARTESIAN_POINT ( 'NONE',  ( -5.200000000000022382, 12.50000000000000000, 0.3464101615137735735 ) ) ;
#19846=CIRCLE ( 'NONE', #93008, 0.06509327318403745899 ) ;
#19847=DIRECTION ( 'NONE',  ( -0.000000000000000000, 1.000000000000000000, -0.000000000000000000 ) ) ;
#19848=ORIENTED_EDGE ( 'NONE', *, *, #5057, .F. ) ;
#19849=EDGE_LOOP ( 'NONE', ( #15029, #50328 ) ) ;
#19850=VERTEX_POINT ( 'NONE', #64246 ) ;
#19851=VERTEX_POINT ( 'NONE', #66176 ) ;
#19852=DIRECTION ( 'NONE',  ( 0.000000000000000000, 1.000000000000000000, 0.000000000000000000 ) ) ;
#19853=CARTESIAN_POINT ( 'NONE',  ( -13.74999999999998757, 12.50000000000000000, 1.407149913249511997 ) ) ;
#19854=ORIENTED_EDGE ( 'NONE', *, *, #21646, .F. ) ;
#19856=ORIENTED_EDGE ( 'NONE', *, *, #106676, .T. ) ;
#19857=FACE_OUTER_BOUND ( 'NONE', #31370, .T. ) ;
#19858=AXIS2_PLACEMENT_3D ( 'NONE', #66346, #125279, #65706 ) ;
#19859=VECTOR ( 'NONE', #9655, 1000.000000000000000 ) ;
#19860=CARTESIAN_POINT ( 'NONE',  ( -12.09999999999999609, 2.500000000000000000, 0.1000000000000017403 ) ) ;
#19861=CARTESIAN_POINT ( 'NONE',  ( 5.649999999999934630, 12.50000000000000000, 6.776507416713035248 ) ) ;
#19862=CARTESIAN_POINT ( 'NONE',  ( -4.350000000000023626, 12.50000000000000000, 2.511473670974873507 ) ) ;
#19863=DIRECTION ( 'NONE',  ( 0.000000000000000000, 1.000000000000000000, 0.000000000000000000 ) ) ;
#19865=DIRECTION ( 'NONE',  ( 0.000000000000000000, 0.000000000000000000, -1.000000000000000000 ) ) ;
#19866=ORIENTED_EDGE ( 'NONE', *, *, #14133, .T. ) ;
#19867=CARTESIAN_POINT ( 'NONE',  ( -0.6500000000000389910, 2.500000000000000000, -6.148780366869526226 ) ) ;
#19868=ORIENTED_EDGE ( 'NONE', *, *, #2323, .F. ) ;
#19869=AXIS2_PLACEMENT_3D ( 'NONE', #127165, #69501, #70802 ) ;
#19870=EDGE_CURVE ( 'NONE', #22721, #11513, #24971, .T. ) ;
#19871=ORIENTED_EDGE ( 'NONE', *, *, #4506, .T. ) ;
#19873=CARTESIAN_POINT ( 'NONE',  ( 1.249999999999952482, 2.500000000000000000, -5.802370205355749988 ) ) ;
#19874=ORIENTED_EDGE ( 'NONE', *, *, #121641, .T. ) ;
#19876=ORIENTED_EDGE ( 'NONE', *, *, #84315, .T. ) ;
#19877=ADVANCED_FACE ( 'NONE', ( #15124 ), #120046, .T. ) ;
#19878=DIRECTION ( 'NONE',  ( -0.000000000000000000, -1.000000000000000000, -0.000000000000000000 ) ) ;
#19879=CARTESIAN_POINT ( 'NONE',  ( -1.850000000000033840, 2.500000000000000000, 2.411473670974873862 ) ) ;
#19880=CIRCLE ( 'NONE', #103497, 0.1000000000000000472 ) ;
#19881=DIRECTION ( 'NONE',  ( -0.000000000000000000, -1.000000000000000000, -0.000000000000000000 ) ) ;
#19882=CONICAL_SURFACE ( 'NONE', #47072, 0.1000000000000002554, 0.003490658503988666988 ) ;
#19883=DIRECTION ( 'NONE',  ( 0.000000000000000000, 0.000000000000000000, -1.000000000000000000 ) ) ;
#19884=EDGE_CURVE ( 'NONE', #19791, #55495, #72028, .T. ) ;
#19885=FACE_OUTER_BOUND ( 'NONE', #84153, .T. ) ;
#19886=EDGE_CURVE ( 'NONE', #81561, #47875, #43983, .T. ) ;
#19887=ADVANCED_FACE ( 'NONE', ( #13853 ), #115918, .T. ) ;
#19888=VERTEX_POINT ( 'NONE', #55079 ) ;
#19889=CARTESIAN_POINT ( 'NONE',  ( -6.450000000000014388, 2.500000000000000000, 1.918653347947321564 ) ) ;
#19890=ORIENTED_EDGE ( 'NONE', *, *, #85311, .F. ) ;
#19891=FACE_OUTER_BOUND ( 'NONE', #54961, .T. ) ;
#19892=EDGE_CURVE ( 'NONE', #34472, #107528, #21859, .T. ) ;
#19893=ORIENTED_EDGE ( 'NONE', *, *, #117850, .F. ) ;
#19895=CARTESIAN_POINT ( 'NONE',  ( 1.649999999999951950, 12.50000000000000000, -5.802370205355749988 ) ) ;
#19896=ORIENTED_EDGE ( 'NONE', *, *, #41928, .T. ) ;
#19897=DIRECTION ( 'NONE',  ( 0.000000000000000000, 0.000000000000000000, 1.000000000000000000 ) ) ;
#19898=DIRECTION ( 'NONE',  ( 0.000000000000000000, 1.000000000000000000, 0.000000000000000000 ) ) ;
#19899=CIRCLE ( 'NONE', #128679, 0.06509327318403745899 ) ;
#19900=ORIENTED_EDGE ( 'NONE', *, *, #21955, .T. ) ;
#19901=ADVANCED_FACE ( 'NONE', ( #54423 ), #94347, .T. ) ;
#19902=CIRCLE ( 'NONE', #9430, 0.1000000000000002554 ) ;
#19903=CONICAL_SURFACE ( 'NONE', #109776, 0.09999999999999982514, 0.003490658503988666988 ) ;
#19904=DIRECTION ( 'NONE',  ( 0.000000000000000000, 1.000000000000000000, 0.000000000000000000 ) ) ;
#19905=EDGE_LOOP ( 'NONE', ( #126154, #21488 ) ) ;
#19906=AXIS2_PLACEMENT_3D ( 'NONE', #12585, #83904, #2124 ) ;
#19908=CARTESIAN_POINT ( 'NONE',  ( 1.849999999999950573, 12.50000000000000000, 2.511473670974873507 ) ) ;
#19909=LINE ( 'NONE', #119373, #65963 ) ;
#19910=DIRECTION ( 'NONE',  ( 0.000000000000000000, -0.000000000000000000, 1.000000000000000000 ) ) ;
#19911=DIRECTION ( 'NONE',  ( 0.000000000000000000, 1.000000000000000000, 0.000000000000000000 ) ) ;
#19912=CARTESIAN_POINT ( 'NONE',  ( 12.69999999999990159, 12.50000000000000000, -4.048810130592463530 ) ) ;
#19913=CONICAL_SURFACE ( 'NONE', #101473, 0.09999999999999982514, 0.003490658503988666988 ) ;
#19914=ORIENTED_EDGE ( 'NONE', *, *, #124164, .T. ) ;
#19915=AXIS2_PLACEMENT_3D ( 'NONE', #25036, #45976, #64944 ) ;
#19916=DIRECTION ( 'NONE',  ( -0.000000000000000000, 1.000000000000000000, -0.000000000000000000 ) ) ;
#19917=AXIS2_PLACEMENT_3D ( 'NONE', #11537, #118918, #61943 ) ;
#19918=EDGE_LOOP ( 'NONE', ( #27382, #128493, #96272, #87917 ) ) ;
#19919=CIRCLE ( 'NONE', #49180, 0.09999999999999982514 ) ;
#19920=CARTESIAN_POINT ( 'NONE',  ( 6.849999999999929479, 2.500000000000000000, 6.248780366869520542 ) ) ;
#19921=DIRECTION ( 'NONE',  ( -0.000000000000000000, 1.000000000000000000, -0.000000000000000000 ) ) ;
#19922=CIRCLE ( 'NONE', #30402, 0.09999999999999999167 ) ;
#19923=CONICAL_SURFACE ( 'NONE', #30404, 0.09999999999999982514, 0.003490658503988666988 ) ;
#19924=CARTESIAN_POINT ( 'NONE',  ( 3.749999999999944045, 2.500000000000000000, -7.188010851410854052 ) ) ;
#19925=CARTESIAN_POINT ( 'NONE',  ( 12.09999999999990195, 12.50000000000000000, -2.276824562219559311E-15 ) ) ;
#19926=DIRECTION ( 'NONE',  ( 0.000000000000000000, -0.9999939076577903929, 0.003490651415223739937 ) ) ;
#19927=CARTESIAN_POINT ( 'NONE',  ( -14.99999999999994671, 2.500000000000000000, 0.000000000000000000 ) ) ;
#19928=PLANE ( 'NONE',  #36987 ) ;
#19929=ORIENTED_EDGE ( 'NONE', *, *, #79605, .F. ) ;
#19930=DIRECTION ( 'NONE',  ( -0.000000000000000000, -1.000000000000000000, -0.000000000000000000 ) ) ;
#19931=EDGE_CURVE ( 'NONE', #57931, #30852, #5097, .T. ) ;
#19932=DIRECTION ( 'NONE',  ( 0.000000000000000000, 0.000000000000000000, 1.000000000000000000 ) ) ;
#19933=CARTESIAN_POINT ( 'NONE',  ( 12.94999999999990337, 2.500000000000000000, 2.265063509461097357 ) ) ;
#19934=CONICAL_SURFACE ( 'NONE', #36671, 0.1000000000000002554, 0.003490658503988666988 ) ;
#19935=ORIENTED_EDGE ( 'NONE', *, *, #115256, .F. ) ;
#19936=DIRECTION ( 'NONE',  ( -0.000000000000000000, 1.000000000000000000, -0.000000000000000000 ) ) ;
#19937=ADVANCED_FACE ( 'NONE', ( #74718 ), #19785, .T. ) ;
#19938=ORIENTED_EDGE ( 'NONE', *, *, #80631, .T. ) ;
#19939=EDGE_LOOP ( 'NONE', ( #122924, #81227 ) ) ;
#19940=LINE ( 'NONE', #938, #23833 ) ;
#19941=AXIS2_PLACEMENT_3D ( 'NONE', #64251, #106116, #104182 ) ;
#19942=ORIENTED_EDGE ( 'NONE', *, *, #43455, .T. ) ;
#19943=CARTESIAN_POINT ( 'NONE',  ( -5.400000000000019895, 12.50000000000000000, 4.265033745738159077 ) ) ;
#19944=DIRECTION ( 'NONE',  ( 0.000000000000000000, 1.000000000000000000, 0.000000000000000000 ) ) ;
#19945=CONICAL_SURFACE ( 'NONE', #57601, 0.1000000000000002554, 0.003490658503988666988 ) ;
#19946=CIRCLE ( 'NONE', #70123, 0.06509327318403745899 ) ;
#19947=EDGE_LOOP ( 'NONE', ( #36102, #4181 ) ) ;
#19948=FACE_OUTER_BOUND ( 'NONE', #15952, .T. ) ;
#19949=CARTESIAN_POINT ( 'NONE',  ( 3.949999999999941558, 2.500000000000000000, -1.818653347947326138 ) ) ;
#19950=CARTESIAN_POINT ( 'NONE',  ( 10.59999999999990905, 2.500000000000000000, -4.083716857408426826 ) ) ;
#19951=ORIENTED_EDGE ( 'NONE', *, *, #4954, .F. ) ;
#19952=CIRCLE ( 'NONE', #28270, 0.06509327318403745899 ) ;
#19953=VERTEX_POINT ( 'NONE', #95011 ) ;
#19954=AXIS2_PLACEMENT_3D ( 'NONE', #110449, #41098, #20792 ) ;
#19955=VERTEX_POINT ( 'NONE', #5322 ) ;
#19956=DIRECTION ( 'NONE',  ( -4.274815082592931898E-19, -0.9999939076577903929, -0.003490651415223739937 ) ) ;
#19957=DIRECTION ( 'NONE',  ( 0.000000000000000000, 1.000000000000000000, 0.000000000000000000 ) ) ;
#19958=CARTESIAN_POINT ( 'NONE',  ( 5.399999999999936406, 12.50000000000000000, -3.572213422710612374 ) ) ;
#19959=FACE_BOUND ( 'NONE', #49605, .T. ) ;
#19960=VERTEX_POINT ( 'NONE', #45267 ) ;
#19961=CARTESIAN_POINT ( 'NONE',  ( 5.449999999999934452, 2.500000000000000000, 2.165063509461097713 ) ) ;
#19962=DIRECTION ( 'NONE',  ( 0.000000000000000000, 1.000000000000000000, 0.000000000000000000 ) ) ;
#19963=EDGE_LOOP ( 'NONE', ( #39598, #124135, #91560, #67490 ) ) ;
#19964=DIRECTION ( 'NONE',  ( 0.000000000000000000, 0.000000000000000000, 1.000000000000000000 ) ) ;
#19965=EDGE_CURVE ( 'NONE', #95189, #60634, #84528, .T. ) ;
#19966=CONICAL_SURFACE ( 'NONE', #78563, 0.09999999999999982514, 0.003490658503988666988 ) ;
#19967=FACE_OUTER_BOUND ( 'NONE', #126411, .T. ) ;
#19968=CONICAL_SURFACE ( 'NONE', #61752, 0.09999999999999982514, 0.003490658503988666988 ) ;
#19969=CARTESIAN_POINT ( 'NONE',  ( 3.149999999999946176, 2.500000000000000000, -6.148780366869526226 ) ) ;
#19970=DIRECTION ( 'NONE',  ( 0.000000000000000000, 0.000000000000000000, 1.000000000000000000 ) ) ;
#19971=PLANE ( 'NONE',  #13102 ) ;
#19972=FACE_OUTER_BOUND ( 'NONE', #70764, .T. ) ;
#19974=EDGE_CURVE ( 'NONE', #92776, #34089, #15785, .T. ) ;
#19975=ORIENTED_EDGE ( 'NONE', *, *, #118115, .F. ) ;
#19976=ORIENTED_EDGE ( 'NONE', *, *, #44728, .T. ) ;
#19977=EDGE_LOOP ( 'NONE', ( #83533, #81975, #9263, #123466 ) ) ;
#19978=AXIS2_PLACEMENT_3D ( 'NONE', #111774, #109173, #10344 ) ;
#19979=ORIENTED_EDGE ( 'NONE', *, *, #54583, .F. ) ;
#19980=ORIENTED_EDGE ( 'NONE', *, *, #51749, .T. ) ;
#19981=DIRECTION ( 'NONE',  ( 0.000000000000000000, 1.000000000000000000, 0.000000000000000000 ) ) ;
#19982=EDGE_CURVE ( 'NONE', #60636, #66637, #96271, .T. ) ;
#19983=DIRECTION ( 'NONE',  ( 0.000000000000000000, 0.000000000000000000, -1.000000000000000000 ) ) ;
#19984=ORIENTED_EDGE ( 'NONE', *, *, #42754, .F. ) ;
#19985=FACE_BOUND ( 'NONE', #81919, .T. ) ;
#19987=VECTOR ( 'NONE', #101981, 1000.000000000000000 ) ;
#19988=FACE_OUTER_BOUND ( 'NONE', #81893, .T. ) ;
#19989=CIRCLE ( 'NONE', #22156, 0.1000000000000000472 ) ;
#19990=EDGE_CURVE ( 'NONE', #125138, #74230, #61647, .T. ) ;
#19991=CARTESIAN_POINT ( 'NONE',  ( 0.3999999999999619971, 12.50000000000000000, -1.084202172485504434E-16 ) ) ;
#19992=CIRCLE ( 'NONE', #126606, 0.06509327318403745899 ) ;
#19993=CARTESIAN_POINT ( 'NONE',  ( 12.04999999999990479, 2.500000000000000000, 2.265063509461097357 ) ) ;
#19994=DIRECTION ( 'NONE',  ( -0.000000000000000000, -1.000000000000000000, -0.000000000000000000 ) ) ;
#19996=DIRECTION ( 'NONE',  ( -0.000000000000000000, -1.000000000000000000, -0.000000000000000000 ) ) ;
#19997=EDGE_CURVE ( 'NONE', #30351, #71261, #40732, .T. ) ;
#19998=DIRECTION ( 'NONE',  ( -0.000000000000000000, 1.000000000000000000, -0.000000000000000000 ) ) ;
#19999=EDGE_LOOP ( 'NONE', ( #74108, #74327 ) ) ;
#20000=CONICAL_SURFACE ( 'NONE', #126612, 0.1000000000000002554, 0.003490658503988666988 ) ;
#20001=ORIENTED_EDGE ( 'NONE', *, *, #106874, .F. ) ;
#20002=ORIENTED_EDGE ( 'NONE', *, *, #106424, .T. ) ;
#20003=VERTEX_POINT ( 'NONE', #118498 ) ;
#20004=ORIENTED_EDGE ( 'NONE', *, *, #2117, .F. ) ;
#20005=ORIENTED_EDGE ( 'NONE', *, *, #65374, .F. ) ;
#20006=VECTOR ( 'NONE', #38283, 1000.000000000000000 ) ;
#20008=DIRECTION ( 'NONE',  ( 0.000000000000000000, 1.000000000000000000, 0.000000000000000000 ) ) ;
#20009=ORIENTED_EDGE ( 'NONE', *, *, #38190, .F. ) ;
#20010=CARTESIAN_POINT ( 'NONE',  ( 6.249999999999968914, 2.500000000000000000, -6.495190528383302464 ) ) ;
#20011=CIRCLE ( 'NONE', #91017, 0.1000000000000002554 ) ;
#20012=DIRECTION ( 'NONE',  ( -0.000000000000000000, -1.000000000000000000, -0.000000000000000000 ) ) ;
#20013=CONICAL_SURFACE ( 'NONE', #93179, 0.09999999999999999167, 0.003490658503988666988 ) ;
#20014=DIRECTION ( 'NONE',  ( 0.000000000000000000, 1.000000000000000000, 0.000000000000000000 ) ) ;
#20016=DIRECTION ( 'NONE',  ( 0.000000000000000000, 0.000000000000000000, 1.000000000000000000 ) ) ;
#20017=DIRECTION ( 'NONE',  ( 0.000000000000000000, 1.000000000000000000, 0.000000000000000000 ) ) ;
#20018=VECTOR ( 'NONE', #11838, 1000.000000000000000 ) ;
#20019=CARTESIAN_POINT ( 'NONE',  ( -13.34999999999999076, 2.500000000000000000, 2.165063509461101265 ) ) ;
#20020=ORIENTED_EDGE ( 'NONE', *, *, #88840, .F. ) ;
#20021=CARTESIAN_POINT ( 'NONE',  ( -12.29999999999999538, 2.500000000000000000, -0.3464101615137741841 ) ) ;
#20022=EDGE_LOOP ( 'NONE', ( #65956, #15152, #98745, #49067 ) ) ;
#20023=EDGE_CURVE ( 'NONE', #52300, #25799, #44634, .T. ) ;
#20024=VERTEX_POINT ( 'NONE', #17042 ) ;
#20025=CARTESIAN_POINT ( 'NONE',  ( -3.950000000000028155, 12.50000000000000000, -6.906693963081115051 ) ) ;
#20026=DIRECTION ( 'NONE',  ( -0.000000000000000000, -1.000000000000000000, -0.000000000000000000 ) ) ;
#20027=CARTESIAN_POINT ( 'NONE',  ( -0.2000000000000404232, 2.500000000000000000, 3.983716857408420964 ) ) ;
#20028=AXIS2_PLACEMENT_3D ( 'NONE', #4497, #54913, #94850 ) ;
#20029=ORIENTED_EDGE ( 'NONE', *, *, #18224, .F. ) ;
#20030=VERTEX_POINT ( 'NONE', #39333 ) ;
#20031=EDGE_CURVE ( 'NONE', #94655, #32380, #58953, .T. ) ;
#20032=CARTESIAN_POINT ( 'NONE',  ( 5.849999999999935696, 12.50000000000000000, -6.495190528383302464 ) ) ;
#20033=CARTESIAN_POINT ( 'NONE',  ( 9.599999999999914380, 12.50000000000000000, 4.957854068765711553 ) ) ;
#20034=DIRECTION ( 'NONE',  ( 0.000000000000000000, 1.000000000000000000, 0.000000000000000000 ) ) ;
#20035=DIRECTION ( 'NONE',  ( -0.000000000000000000, -1.000000000000000000, -0.000000000000000000 ) ) ;
#20036=EDGE_LOOP ( 'NONE', ( #97838, #87852, #44093, #23758 ) ) ;
#20037=ADVANCED_FACE ( 'NONE', ( #117842 ), #90589, .T. ) ;
#20038=LINE ( 'NONE', #118225, #79532 ) ;
#20039=CIRCLE ( 'NONE', #26299, 0.1000000000000002554 ) ;
#20040=EDGE_CURVE ( 'NONE', #2801, #27444, #17706, .T. ) ;
#20041=VECTOR ( 'NONE', #77437, 1000.000000000000000 ) ;
#20042=EDGE_CURVE ( 'NONE', #28525, #53869, #21652, .T. ) ;
#20043=EDGE_LOOP ( 'NONE', ( #102926, #47898, #111579, #61654 ) ) ;
#20044=LINE ( 'NONE', #99891, #1836 ) ;
#20045=AXIS2_PLACEMENT_3D ( 'NONE', #59917, #58614, #22565 ) ;
#20046=EDGE_LOOP ( 'NONE', ( #79737, #10232 ) ) ;
#20047=CIRCLE ( 'NONE', #61909, 0.09999999999999999167 ) ;
#20048=CARTESIAN_POINT ( 'NONE',  ( 8.099999999999923261, 2.500000000000000000, -4.083716857408426826 ) ) ;
#20049=EDGE_CURVE ( 'NONE', #85597, #91594, #7898, .T. ) ;
#20050=FACE_OUTER_BOUND ( 'NONE', #38631, .T. ) ;
#20052=DIRECTION ( 'NONE',  ( -0.000000000000000000, 1.000000000000000000, -0.000000000000000000 ) ) ;
#20053=ORIENTED_EDGE ( 'NONE', *, *, #112275, .T. ) ;
#20054=EDGE_CURVE ( 'NONE', #62991, #118696, #5188, .T. ) ;
#20055=CONICAL_SURFACE ( 'NONE', #120395, 0.1000000000000002554, 0.003490658503988666988 ) ;
#20056=LINE ( 'NONE', #21999, #21731 ) ;
#20057=ADVANCED_FACE ( 'NONE', ( #68757 ), #46983, .T. ) ;
#20058=CIRCLE ( 'NONE', #24250, 0.1000000000000000472 ) ;
#20059=CIRCLE ( 'NONE', #116172, 0.06509327318403745899 ) ;
#20060=ORIENTED_EDGE ( 'NONE', *, *, #89382, .T. ) ;
#20061=ORIENTED_EDGE ( 'NONE', *, *, #33345, .T. ) ;
#20062=CARTESIAN_POINT ( 'NONE',  ( -12.04999999999999716, 12.50000000000000000, -2.230156782645135394 ) ) ;
#20063=DIRECTION ( 'NONE',  ( 0.000000000000000000, -0.9999939076577903929, 0.003490651415223739937 ) ) ;
#20064=CARTESIAN_POINT ( 'NONE',  ( -4.150000000000025224, 12.50000000000000000, -1.472243186433550122 ) ) ;
#20066=CARTESIAN_POINT ( 'NONE',  ( 7.299999999999927880, 2.500000000000000000, 4.083716857408421497 ) ) ;
#20067=FACE_OUTER_BOUND ( 'NONE', #45786, .T. ) ;
#20068=VECTOR ( 'NONE', #125122, 1000.000000000000000 ) ;
#20069=LINE ( 'NONE', #80918, #42732 ) ;
#20070=LINE ( 'NONE', #110990, #47025 ) ;
#20071=DIRECTION ( 'NONE',  ( -0.000000000000000000, -1.000000000000000000, -0.000000000000000000 ) ) ;
#20072=ORIENTED_EDGE ( 'NONE', *, *, #111544, .F. ) ;
#20073=DIRECTION ( 'NONE',  ( 0.000000000000000000, 1.000000000000000000, 0.000000000000000000 ) ) ;
#20074=FACE_OUTER_BOUND ( 'NONE', #108974, .T. ) ;
#20075=DIRECTION ( 'NONE',  ( 0.000000000000000000, 0.000000000000000000, 1.000000000000000000 ) ) ;
#20076=CARTESIAN_POINT ( 'NONE',  ( -7.100000000000017408, 12.50000000000000000, -3.637306695894650055 ) ) ;
#20077=FACE_OUTER_BOUND ( 'NONE', #63138, .T. ) ;
#20078=EDGE_LOOP ( 'NONE', ( #106370, #21078 ) ) ;
#20079=DIRECTION ( 'NONE',  ( 0.000000000000000000, -0.9999939076577903929, 0.003490651415223739937 ) ) ;
#20080=CONICAL_SURFACE ( 'NONE', #59822, 0.09999999999999999167, 0.003490658503988666988 ) ;
#20081=EDGE_CURVE ( 'NONE', #96072, #46924, #111826, .T. ) ;
#20082=AXIS2_PLACEMENT_3D ( 'NONE', #62893, #21686, #32162 ) ;
#20083=CARTESIAN_POINT ( 'NONE',  ( 1.849999999999950573, 2.500000000000000000, 2.611473670974873151 ) ) ;
#20084=CARTESIAN_POINT ( 'NONE',  ( 0.3999999999999628852, 2.500000000000000000, 0.7928203230275517877 ) ) ;
#20085=ORIENTED_EDGE ( 'NONE', *, *, #89308, .F. ) ;
#20086=ORIENTED_EDGE ( 'NONE', *, *, #126692, .F. ) ;
#20087=AXIS2_PLACEMENT_3D ( 'NONE', #71150, #109125, #129463 ) ;
#20088=DIRECTION ( 'NONE',  ( -0.000000000000000000, 1.000000000000000000, -0.000000000000000000 ) ) ;
#20089=EDGE_CURVE ( 'NONE', #89954, #48809, #88529, .T. ) ;
#20090=EDGE_LOOP ( 'NONE', ( #45943, #86642, #53501, #6429 ) ) ;
#20091=ORIENTED_EDGE ( 'NONE', *, *, #99667, .T. ) ;
#20092=CARTESIAN_POINT ( 'NONE',  ( -6.250000000000015987, 2.500000000000000000, 5.802370205355744659 ) ) ;
#20094=CARTESIAN_POINT ( 'NONE',  ( 9.599999999999914380, 2.500000000000000000, 4.430127018922196847 ) ) ;
#20095=VECTOR ( 'NONE', #105552, 1000.000000000000000 ) ;
#20096=DIRECTION ( 'NONE',  ( -0.000000000000000000, 1.000000000000000000, -0.000000000000000000 ) ) ;
#20097=ORIENTED_EDGE ( 'NONE', *, *, #62845, .T. ) ;
#20098=AXIS2_PLACEMENT_3D ( 'NONE', #84573, #74758, #63656 ) ;
#20099=DIRECTION ( 'NONE',  ( 0.000000000000000000, 0.000000000000000000, -1.000000000000000000 ) ) ;
#20100=VERTEX_POINT ( 'NONE', #127678 ) ;
#20102=DIRECTION ( 'NONE',  ( -0.000000000000000000, -1.000000000000000000, -0.000000000000000000 ) ) ;
#20103=FACE_OUTER_BOUND ( 'NONE', #14264, .T. ) ;
#20104=ORIENTED_EDGE ( 'NONE', *, *, #70522, .F. ) ;
#20105=VERTEX_POINT ( 'NONE', #79242 ) ;
#20106=ORIENTED_EDGE ( 'NONE', *, *, #341, .T. ) ;
#20107=ORIENTED_EDGE ( 'NONE', *, *, #82061, .F. ) ;
#20108=EDGE_LOOP ( 'NONE', ( #93169, #2353 ) ) ;
#20110=CARTESIAN_POINT ( 'NONE',  ( 1.699999999999950218, 2.500000000000000000, 4.230127018922196669 ) ) ;
#20111=FACE_OUTER_BOUND ( 'NONE', #37115, .T. ) ;
#20112=FACE_BOUND ( 'NONE', #27970, .T. ) ;
#20113=DIRECTION ( 'NONE',  ( 0.000000000000000000, -0.000000000000000000, 1.000000000000000000 ) ) ;
#20114=AXIS2_PLACEMENT_3D ( 'NONE', #62818, #83742, #101450 ) ;
#20116=LINE ( 'NONE', #60063, #51106 ) ;
#20117=DIRECTION ( 'NONE',  ( -4.274815082592931898E-19, -0.9999939076577903929, -0.003490651415223739937 ) ) ;
#20119=DIRECTION ( 'NONE',  ( 0.000000000000000000, 0.000000000000000000, -1.000000000000000000 ) ) ;
#20121=DIRECTION ( 'NONE',  ( -0.000000000000000000, 1.000000000000000000, -0.000000000000000000 ) ) ;
#20122=CARTESIAN_POINT ( 'NONE',  ( 13.74999999999993427, 2.500000000000000000, 2.165063509461097713 ) ) ;
#20123=AXIS2_PLACEMENT_3D ( 'NONE', #90142, #121545, #19484 ) ;
#20124=CIRCLE ( 'NONE', #91229, 0.1000000000000002554 ) ;
#20125=EDGE_CURVE ( 'NONE', #13873, #89102, #36745, .T. ) ;
#20126=CARTESIAN_POINT ( 'NONE',  ( 8.949999999999915801, 12.50000000000000000, 6.841600689897072485 ) ) ;
#20127=ORIENTED_EDGE ( 'NONE', *, *, #64344, .T. ) ;
#20128=ORIENTED_EDGE ( 'NONE', *, *, #38799, .F. ) ;
#20129=ORIENTED_EDGE ( 'NONE', *, *, #92792, .T. ) ;
#20130=ORIENTED_EDGE ( 'NONE', *, *, #81802, .F. ) ;
#20131=FACE_OUTER_BOUND ( 'NONE', #107303, .T. ) ;
#20132=ADVANCED_FACE ( 'NONE', ( #18365 ), #14978, .F. ) ;
#20133=DIRECTION ( 'NONE',  ( 0.000000000000000000, -0.000000000000000000, 1.000000000000000000 ) ) ;
#20134=FACE_BOUND ( 'NONE', #89518, .T. ) ;
#20135=ADVANCED_FACE ( 'NONE', ( #122230 ), #78380, .T. ) ;
#20136=CIRCLE ( 'NONE', #93294, 0.1000000000000000472 ) ;
#20137=DIRECTION ( 'NONE',  ( 0.000000000000000000, 0.000000000000000000, 1.000000000000000000 ) ) ;
#20138=AXIS2_PLACEMENT_3D ( 'NONE', #78479, #119656, #128875 ) ;
#20139=VECTOR ( 'NONE', #31436, 1000.000000000000000 ) ;
#20140=EDGE_CURVE ( 'NONE', #81254, #78428, #11170, .T. ) ;
#20141=EDGE_CURVE ( 'NONE', #117403, #71756, #78078, .T. ) ;
#20142=VERTEX_POINT ( 'NONE', #42375 ) ;
#20143=CARTESIAN_POINT ( 'NONE',  ( -5.650000000000019895, 2.500000000000000000, 6.248780366869520542 ) ) ;
#20144=DIRECTION ( 'NONE',  ( 0.000000000000000000, -0.000000000000000000, 1.000000000000000000 ) ) ;
#20145=CARTESIAN_POINT ( 'NONE',  ( -3.749999999999991118, 2.500000000000000000, 2.265063509461097357 ) ) ;
#20146=EDGE_CURVE ( 'NONE', #64905, #101430, #109984, .T. ) ;
#20147=FACE_OUTER_BOUND ( 'NONE', #13145, .T. ) ;
#20149=CARTESIAN_POINT ( 'NONE',  ( 6.849999999999930367, 2.500000000000000000, -6.741600689897078169 ) ) ;
#20150=VERTEX_POINT ( 'NONE', #63292 ) ;
#20151=ORIENTED_EDGE ( 'NONE', *, *, #16884, .T. ) ;
#20152=DIRECTION ( 'NONE',  ( -4.274815082592931898E-19, -0.9999939076577903929, -0.003490651415223739937 ) ) ;
#20153=DIRECTION ( 'NONE',  ( 0.000000000000000000, 1.000000000000000000, 0.000000000000000000 ) ) ;
#20154=ORIENTED_EDGE ( 'NONE', *, *, #121793, .F. ) ;
#20155=DIRECTION ( 'NONE',  ( -0.000000000000000000, -1.000000000000000000, -0.000000000000000000 ) ) ;
#20156=CARTESIAN_POINT ( 'NONE',  ( 4.549999999999935874, 2.500000000000000000, 6.595190528383296780 ) ) ;
#20157=DIRECTION ( 'NONE',  ( 0.000000000000000000, 0.000000000000000000, 1.000000000000000000 ) ) ;
#20158=ORIENTED_EDGE ( 'NONE', *, *, #29732, .T. ) ;
#20159=CARTESIAN_POINT ( 'NONE',  ( 2.499999999999983569, 12.50000000000000000, -2.276824562219559311E-15 ) ) ;
#20160=VERTEX_POINT ( 'NONE', #9843 ) ;
#20161=DIRECTION ( 'NONE',  ( 0.000000000000000000, -0.9999939076577903929, 0.003490651415223739937 ) ) ;
#20162=CIRCLE ( 'NONE', #89211, 0.06509327318403745899 ) ;
#20163=ORIENTED_EDGE ( 'NONE', *, *, #31031, .F. ) ;
#20164=AXIS2_PLACEMENT_3D ( 'NONE', #88976, #128931, #122316 ) ;
#20166=VERTEX_POINT ( 'NONE', #20313 ) ;
#20167=DIRECTION ( 'NONE',  ( -0.000000000000000000, -1.000000000000000000, -0.000000000000000000 ) ) ;
#20168=FACE_OUTER_BOUND ( 'NONE', #112177, .T. ) ;
#20169=FACE_OUTER_BOUND ( 'NONE', #17298, .T. ) ;
#20170=CARTESIAN_POINT ( 'NONE',  ( 10.64999999999990976, 12.50000000000000000, -6.083687093685488989 ) ) ;
#20171=CARTESIAN_POINT ( 'NONE',  ( 15.19999999999989271, 2.500000000000000000, -0.3464101615137783474 ) ) ;
#20172=EDGE_LOOP ( 'NONE', ( #115003, #15706 ) ) ;
#20173=CIRCLE ( 'NONE', #41125, 0.1000000000000002554 ) ;
#20174=ORIENTED_EDGE ( 'NONE', *, *, #20354, .T. ) ;
#20175=EDGE_LOOP ( 'NONE', ( #117069, #2772 ) ) ;
#20176=DIRECTION ( 'NONE',  ( 0.000000000000000000, 0.000000000000000000, -1.000000000000000000 ) ) ;
#20177=DIRECTION ( 'NONE',  ( 0.000000000000000000, 0.000000000000000000, 1.000000000000000000 ) ) ;
#20178=CARTESIAN_POINT ( 'NONE',  ( -2.500000000000030642, 2.500000000000000000, -0.7928203230275542301 ) ) ;
#20179=ADVANCED_FACE ( 'NONE', ( #24666 ), #93404, .T. ) ;
#20180=ORIENTED_EDGE ( 'NONE', *, *, #120229, .F. ) ;
#20181=EDGE_LOOP ( 'NONE', ( #81629, #39152, #9003, #55222 ) ) ;
#20182=EDGE_LOOP ( 'NONE', ( #19781, #113688, #116455, #36198 ) ) ;
#20183=EDGE_CURVE ( 'NONE', #124893, #96482, #50898, .T. ) ;
#20184=CARTESIAN_POINT ( 'NONE',  ( -8.750000000000008882, 2.500000000000000000, 1.572243186433545548 ) ) ;
#20185=EDGE_CURVE ( 'NONE', #99762, #7788, #124341, .T. ) ;
#20186=AXIS2_PLACEMENT_3D ( 'NONE', #73997, #13773, #123101 ) ;
#20187=CIRCLE ( 'NONE', #80834, 0.1000000000000002554 ) ;
#20188=ORIENTED_EDGE ( 'NONE', *, *, #112422, .T. ) ;
#20189=PLANE ( 'NONE',  #27653 ) ;
#20190=AXIS2_PLACEMENT_3D ( 'NONE', #62846, #83145, #92962 ) ;
#20191=CARTESIAN_POINT ( 'NONE',  ( 1.049999999999954525, 12.50000000000000000, -2.511473670974877948 ) ) ;
#20192=CARTESIAN_POINT ( 'NONE',  ( -8.150000000000014566, 2.500000000000000000, -6.248780366869521430 ) ) ;
#20193=DIRECTION ( 'NONE',  ( 0.000000000000000000, 1.000000000000000000, 0.000000000000000000 ) ) ;
#20194=CARTESIAN_POINT ( 'NONE',  ( 14.39999999999989555, 12.50000000000000000, -0.2813168883297408329 ) ) ;
#20196=EDGE_CURVE ( 'NONE', #47163, #110508, #120139, .T. ) ;
#20197=EDGE_CURVE ( 'NONE', #59583, #93582, #84629, .T. ) ;
#20198=DIRECTION ( 'NONE',  ( -1.000000000000000000, 0.000000000000000000, 0.000000000000000000 ) ) ;
#20199=EDGE_CURVE ( 'NONE', #13310, #113079, #124145, .T. ) ;
#20200=ORIENTED_EDGE ( 'NONE', *, *, #341, .F. ) ;
#20201=EDGE_CURVE ( 'NONE', #43211, #112979, #7235, .T. ) ;
#20202=ORIENTED_EDGE ( 'NONE', *, *, #76457, .F. ) ;
#20203=CARTESIAN_POINT ( 'NONE',  ( -12.29999999999999716, 2.500000000000000000, 0.2464101615137776757 ) ) ;
#20204=EDGE_CURVE ( 'NONE', #26160, #1788, #113876, .T. ) ;
#20205=ORIENTED_EDGE ( 'NONE', *, *, #43829, .T. ) ;
#20206=ORIENTED_EDGE ( 'NONE', *, *, #122870, .F. ) ;
#20208=DIRECTION ( 'NONE',  ( 0.000000000000000000, -0.9999939076577903929, 0.003490651415223739937 ) ) ;
#20209=CIRCLE ( 'NONE', #22280, 0.06509327318403745899 ) ;
#20210=CARTESIAN_POINT ( 'NONE',  ( -3.100000000000028511, 12.50000000000000000, -4.611443907251939756 ) ) ;
#20211=EDGE_CURVE ( 'NONE', #45293, #114782, #32135, .T. ) ;
#20212=AXIS2_PLACEMENT_3D ( 'NONE', #117352, #49322, #78119 ) ;
#20213=CARTESIAN_POINT ( 'NONE',  ( 15.59999999999988951, 12.50000000000000000, 0.2813168883297361700 ) ) ;
#20214=DIRECTION ( 'NONE',  ( -0.000000000000000000, -1.000000000000000000, -0.000000000000000000 ) ) ;
#20215=CIRCLE ( 'NONE', #15983, 0.1000000000000002554 ) ;
#20216=CARTESIAN_POINT ( 'NONE',  ( -8.750000000000008882, 2.500000000000000000, 1.472243186433545459 ) ) ;
#20217=CARTESIAN_POINT ( 'NONE',  ( 9.149999999999920419, 12.50000000000000000, -7.188010851410854052 ) ) ;
#20218=AXIS2_PLACEMENT_3D ( 'NONE', #24009, #83583, #35135 ) ;
#20219=CIRCLE ( 'NONE', #74683, 0.06509327318403745899 ) ;
#20220=DIRECTION ( 'NONE',  ( -0.000000000000000000, -1.000000000000000000, -0.000000000000000000 ) ) ;
#20221=VERTEX_POINT ( 'NONE', #84212 ) ;
#20222=AXIS2_PLACEMENT_3D ( 'NONE', #66641, #107216, #85645 ) ;
#20223=EDGE_LOOP ( 'NONE', ( #91936, #128985, #79393, #115592 ) ) ;
#20224=VERTEX_POINT ( 'NONE', #52829 ) ;
#20225=AXIS2_PLACEMENT_3D ( 'NONE', #34017, #64115, #114499 ) ;
#20226=ORIENTED_EDGE ( 'NONE', *, *, #95489, .T. ) ;
#20227=CARTESIAN_POINT ( 'NONE',  ( -14.39999999999998614, 12.50000000000000000, 0.2813168883297384459 ) ) ;
#20228=CARTESIAN_POINT ( 'NONE',  ( 11.64999999999990443, 12.50000000000000000, 2.792790559304612064 ) ) ;
#20229=VECTOR ( 'NONE', #31869, 1000.000000000000000 ) ;
#20230=ORIENTED_EDGE ( 'NONE', *, *, #55766, .F. ) ;
#20231=DIRECTION ( 'NONE',  ( -0.000000000000000000, -1.000000000000000000, -0.000000000000000000 ) ) ;
#20232=CARTESIAN_POINT ( 'NONE',  ( -6.249999999999981348, 2.500000000000000000, 6.495190528383297135 ) ) ;
#20233=AXIS2_PLACEMENT_3D ( 'NONE', #99885, #128724, #59332 ) ;
#20234=AXIS2_PLACEMENT_3D ( 'NONE', #53787, #123805, #95650 ) ;
#20235=CARTESIAN_POINT ( 'NONE',  ( 3.549999999999940314, 2.500000000000000000, 6.741600689897071952 ) ) ;
#20236=CARTESIAN_POINT ( 'NONE',  ( 15.39999999999989022, 2.500000000000000000, -2.385244779468109755E-15 ) ) ;
#20237=ORIENTED_EDGE ( 'NONE', *, *, #26631, .F. ) ;
#20238=CARTESIAN_POINT ( 'NONE',  ( 4.149999999999941735, 2.500000000000000000, -5.902370205355750521 ) ) ;
#20239=DIRECTION ( 'NONE',  ( 0.000000000000000000, 0.000000000000000000, 1.000000000000000000 ) ) ;
#20240=ORIENTED_EDGE ( 'NONE', *, *, #46855, .T. ) ;
#20241=EDGE_CURVE ( 'NONE', #7975, #118333, #48850, .T. ) ;
#20242=EDGE_LOOP ( 'NONE', ( #20494, #91539, #65000, #126350 ) ) ;
#20243=ORIENTED_EDGE ( 'NONE', *, *, #36845, .F. ) ;
#20244=ORIENTED_EDGE ( 'NONE', *, *, #58988, .F. ) ;
#20245=DIRECTION ( 'NONE',  ( 0.000000000000000000, 0.000000000000000000, 1.000000000000000000 ) ) ;
#20246=AXIS2_PLACEMENT_3D ( 'NONE', #24676, #25292, #24037 ) ;
#20247=DIRECTION ( 'NONE',  ( 0.000000000000000000, 0.000000000000000000, -1.000000000000000000 ) ) ;
#20248=FACE_OUTER_BOUND ( 'NONE', #25470, .T. ) ;
#20249=CARTESIAN_POINT ( 'NONE',  ( 3.549999999999942979, 2.500000000000000000, 1.818653347947321475 ) ) ;
#20250=ORIENTED_EDGE ( 'NONE', *, *, #35826, .F. ) ;
#20251=DIRECTION ( 'NONE',  ( 0.000000000000000000, 0.000000000000000000, 1.000000000000000000 ) ) ;
#20252=DIRECTION ( 'NONE',  ( 0.000000000000000000, 1.000000000000000000, 0.000000000000000000 ) ) ;
#20253=DIRECTION ( 'NONE',  ( -0.000000000000000000, -1.000000000000000000, -0.000000000000000000 ) ) ;
#20254=FACE_OUTER_BOUND ( 'NONE', #28019, .T. ) ;
#20255=ORIENTED_EDGE ( 'NONE', *, *, #57417, .F. ) ;
#20256=CIRCLE ( 'NONE', #110143, 0.06509327318403745899 ) ;
#20258=AXIS2_PLACEMENT_3D ( 'NONE', #27792, #919, #57921 ) ;
#20259=EDGE_LOOP ( 'NONE', ( #48934, #105451, #18596, #40704 ) ) ;
#20260=VERTEX_POINT ( 'NONE', #112405 ) ;
#20261=DIRECTION ( 'NONE',  ( 0.000000000000000000, 0.000000000000000000, 1.000000000000000000 ) ) ;
#20262=DIRECTION ( 'NONE',  ( -0.000000000000000000, 1.000000000000000000, -0.000000000000000000 ) ) ;
#20263=FACE_BOUND ( 'NONE', #50859, .T. ) ;
#20264=DIRECTION ( 'NONE',  ( 0.000000000000000000, 1.000000000000000000, 0.000000000000000000 ) ) ;
#20265=CARTESIAN_POINT ( 'NONE',  ( 9.999999999999911182, 2.500000000000000000, -3.637306695894650055 ) ) ;
#20266=AXIS2_PLACEMENT_3D ( 'NONE', #13509, #43017, #103191 ) ;
#20267=CARTESIAN_POINT ( 'NONE',  ( 9.399999999999915090, 2.500000000000000000, 4.576537180435972019 ) ) ;
#20268=FACE_OUTER_BOUND ( 'NONE', #61761, .T. ) ;
#20269=CARTESIAN_POINT ( 'NONE',  ( 7.699999999999925571, 12.50000000000000000, -4.676537180435978769 ) ) ;
#20270=CARTESIAN_POINT ( 'NONE',  ( -9.400000000000009237, 2.500000000000000000, -3.983716857408421852 ) ) ;
#20271=DIRECTION ( 'NONE',  ( 0.000000000000000000, 1.000000000000000000, 0.000000000000000000 ) ) ;
#20272=VERTEX_POINT ( 'NONE', #33831 ) ;
#20273=AXIS2_PLACEMENT_3D ( 'NONE', #75275, #89451, #18122 ) ;
#20274=CONICAL_SURFACE ( 'NONE', #68292, 0.09999999999999982514, 0.003490658503988666988 ) ;
#20275=CARTESIAN_POINT ( 'NONE',  ( 2.499999999999947153, 2.500000000000000000, 3.637306695894644726 ) ) ;
#20276=CONICAL_SURFACE ( 'NONE', #97641, 0.1000000000000000472, 0.003490658503988666988 ) ;
#20277=EDGE_CURVE ( 'NONE', #90767, #91316, #101362, .T. ) ;
#20278=DIRECTION ( 'NONE',  ( -0.000000000000000000, 1.000000000000000000, -0.000000000000000000 ) ) ;
#20279=VERTEX_POINT ( 'NONE', #24024 ) ;
#20280=ORIENTED_EDGE ( 'NONE', *, *, #40138, .F. ) ;
#20281=CARTESIAN_POINT ( 'NONE',  ( 12.94999999999989981, 2.500000000000000000, -2.265063509461101798 ) ) ;
#20282=EDGE_CURVE ( 'NONE', #102223, #128465, #23990, .T. ) ;
#20283=DIRECTION ( 'NONE',  ( 0.000000000000000000, 1.000000000000000000, 0.000000000000000000 ) ) ;
#20284=FACE_BOUND ( 'NONE', #56062, .T. ) ;
#20285=EDGE_CURVE ( 'NONE', #111104, #63288, #34504, .T. ) ;
#20286=DIRECTION ( 'NONE',  ( 0.000000000000000000, 1.000000000000000000, 0.000000000000000000 ) ) ;
#20287=DIRECTION ( 'NONE',  ( 0.000000000000000000, 0.000000000000000000, 1.000000000000000000 ) ) ;
#20288=EDGE_CURVE ( 'NONE', #66014, #115619, #75053, .T. ) ;
#20289=EDGE_CURVE ( 'NONE', #31251, #63386, #55100, .T. ) ;
#20290=VERTEX_POINT ( 'NONE', #104502 ) ;
#20291=DIRECTION ( 'NONE',  ( -0.000000000000000000, -1.000000000000000000, -0.000000000000000000 ) ) ;
#20292=ADVANCED_FACE ( 'NONE', ( #86131 ), #71827, .T. ) ;
#20293=ADVANCED_FACE ( 'NONE', ( #36436 ), #106439, .T. ) ;
#20295=CIRCLE ( 'NONE', #53649, 0.09999999999999982514 ) ;
#20296=ADVANCED_FACE ( 'NONE', ( #115599 ), #92757, .T. ) ;
#20297=AXIS2_PLACEMENT_3D ( 'NONE', #61547, #22908, #83120 ) ;
#20298=EDGE_LOOP ( 'NONE', ( #119954, #12001, #108596, #49931 ) ) ;
#20299=DIRECTION ( 'NONE',  ( 0.000000000000000000, 0.000000000000000000, -1.000000000000000000 ) ) ;
#20300=AXIS2_PLACEMENT_3D ( 'NONE', #81969, #102892, #91799 ) ;
#20301=DIRECTION ( 'NONE',  ( 0.000000000000000000, 0.000000000000000000, 1.000000000000000000 ) ) ;
#20302=CARTESIAN_POINT ( 'NONE',  ( -4.150000000000024336, 2.500000000000000000, -2.757883832488654097 ) ) ;
#20303=DIRECTION ( 'NONE',  ( 0.000000000000000000, -0.000000000000000000, 1.000000000000000000 ) ) ;
#20304=EDGE_CURVE ( 'NONE', #43675, #112383, #30072, .T. ) ;
#20305=CIRCLE ( 'NONE', #110196, 0.06509327318403745899 ) ;
#20306=CONICAL_SURFACE ( 'NONE', #9836, 0.1000000000000002554, 0.003490658503988666988 ) ;
#20307=ADVANCED_FACE ( 'NONE', ( #124800 ), #82294, .T. ) ;
#20308=VERTEX_POINT ( 'NONE', #56673 ) ;
#20309=AXIS2_PLACEMENT_3D ( 'NONE', #117947, #28296, #87198 ) ;
#20310=DIRECTION ( 'NONE',  ( 0.000000000000000000, 0.000000000000000000, -1.000000000000000000 ) ) ;
#20311=DIRECTION ( 'NONE',  ( 0.000000000000000000, 1.000000000000000000, 0.000000000000000000 ) ) ;
#20312=DIRECTION ( 'NONE',  ( 0.000000000000000000, 0.000000000000000000, 1.000000000000000000 ) ) ;
#20313=CARTESIAN_POINT ( 'NONE',  ( 8.749999999999957367, 2.500000000000000000, -6.395190528383301931 ) ) ;
#20314=ORIENTED_EDGE ( 'NONE', *, *, #129182, .T. ) ;
#20315=ORIENTED_EDGE ( 'NONE', *, *, #61461, .T. ) ;
#20316=CIRCLE ( 'NONE', #93480, 0.06509327318403745899 ) ;
#20317=CARTESIAN_POINT ( 'NONE',  ( 5.399999999999934630, 2.500000000000000000, -0.6928203230275542523 ) ) ;
#20318=CIRCLE ( 'NONE', #122531, 0.06509327318403745899 ) ;
#20319=ORIENTED_EDGE ( 'NONE', *, *, #60685, .F. ) ;
#20320=DIRECTION ( 'NONE',  ( 0.000000000000000000, 1.000000000000000000, 0.000000000000000000 ) ) ;
#20321=DIRECTION ( 'NONE',  ( -0.000000000000000000, -1.000000000000000000, -0.000000000000000000 ) ) ;
#20322=CIRCLE ( 'NONE', #35014, 0.09999999999999982514 ) ;
#20323=AXIS2_PLACEMENT_3D ( 'NONE', #102566, #122232, #22753 ) ;
#20324=DIRECTION ( 'NONE',  ( -0.000000000000000000, -1.000000000000000000, -0.000000000000000000 ) ) ;
#20325=ORIENTED_EDGE ( 'NONE', *, *, #112312, .F. ) ;
#20326=LINE ( 'NONE', #97588, #55804 ) ;
#20327=DIRECTION ( 'NONE',  ( -0.000000000000000000, 1.000000000000000000, -0.000000000000000000 ) ) ;
#20328=CARTESIAN_POINT ( 'NONE',  ( -10.00000000000000533, 2.500000000000000000, -5.122947341949750211 ) ) ;
#20329=DIRECTION ( 'NONE',  ( -4.274815082592931898E-19, -0.9999939076577903929, -0.003490651415223739937 ) ) ;
#20330=CARTESIAN_POINT ( 'NONE',  ( 11.24999999999991118, 2.500000000000000000, -2.757883832488654097 ) ) ;
#20331=DIRECTION ( 'NONE',  ( 0.000000000000000000, 1.000000000000000000, 0.000000000000000000 ) ) ;
#20332=ORIENTED_EDGE ( 'NONE', *, *, #91826, .F. ) ;
#20333=VERTEX_POINT ( 'NONE', #126733 ) ;
#20334=DIRECTION ( 'NONE',  ( 0.000000000000000000, 1.000000000000000000, 0.000000000000000000 ) ) ;
#20335=EDGE_LOOP ( 'NONE', ( #116614, #108653 ) ) ;
#20336=FACE_OUTER_BOUND ( 'NONE', #54629, .T. ) ;
#20337=ORIENTED_EDGE ( 'NONE', *, *, #52347, .T. ) ;
#20338=ORIENTED_EDGE ( 'NONE', *, *, #37525, .T. ) ;
#20339=VERTEX_POINT ( 'NONE', #87435 ) ;
#20340=EDGE_CURVE ( 'NONE', #115126, #71852, #109470, .T. ) ;
#20341=AXIS2_PLACEMENT_3D ( 'NONE', #8647, #47315, #48603 ) ;
#20342=CARTESIAN_POINT ( 'NONE',  ( 87.50000000000001421, -3.413194297214860118, -6.711110875543777610 ) ) ;
#20343=ADVANCED_FACE ( 'NONE', ( #95979 ), #6920, .T. ) ;
#20344=DIRECTION ( 'NONE',  ( -0.000000000000000000, 1.000000000000000000, -0.000000000000000000 ) ) ;
#20345=DIRECTION ( 'NONE',  ( -0.000000000000000000, -1.000000000000000000, -0.000000000000000000 ) ) ;
#20346=EDGE_CURVE ( 'NONE', #32403, #27815, #103211, .T. ) ;
#20347=DIRECTION ( 'NONE',  ( 0.000000000000000000, 0.000000000000000000, 1.000000000000000000 ) ) ;
#20348=CARTESIAN_POINT ( 'NONE',  ( -5.850000000000018296, 12.50000000000000000, 1.472243186433545459 ) ) ;
#20349=CARTESIAN_POINT ( 'NONE',  ( -15.19999999999998330, 2.500000000000000000, 0.3464101615137758494 ) ) ;
#20350=LINE ( 'NONE', #100201, #47091 ) ;
#20351=CARTESIAN_POINT ( 'NONE',  ( -5.650000000000023448, 2.500000000000000000, -2.511473670974877948 ) ) ;
#20352=EDGE_CURVE ( 'NONE', #86066, #75789, #86796, .T. ) ;
#20353=CARTESIAN_POINT ( 'NONE',  ( 13.54999999999989946, 12.50000000000000000, 2.511473670974873507 ) ) ;
#20354=EDGE_CURVE ( 'NONE', #47249, #9122, #97264, .T. ) ;
#20355=ORIENTED_EDGE ( 'NONE', *, *, #117958, .F. ) ;
#20356=VECTOR ( 'NONE', #15886, 1000.000000000000000 ) ;
#20357=EDGE_CURVE ( 'NONE', #28403, #42353, #17517, .T. ) ;
#20358=LINE ( 'NONE', #2625, #113408 ) ;
#20359=ORIENTED_EDGE ( 'NONE', *, *, #42994, .T. ) ;
#20360=ORIENTED_EDGE ( 'NONE', *, *, #67693, .F. ) ;
#20361=CARTESIAN_POINT ( 'NONE',  ( 4.149999999999938183, 12.50000000000000000, 7.188010851410848723 ) ) ;
#20362=CARTESIAN_POINT ( 'NONE',  ( -1.450000000000036371, 12.50000000000000000, 6.841600689897072485 ) ) ;
#20364=AXIS2_PLACEMENT_3D ( 'NONE', #108466, #90103, #48926 ) ;
#20365=CIRCLE ( 'NONE', #122770, 0.06509327318403745899 ) ;
#20367=AXIS2_PLACEMENT_3D ( 'NONE', #100990, #51273, #42753 ) ;
#20368=DIRECTION ( 'NONE',  ( 0.000000000000000000, 1.000000000000000000, 0.000000000000000000 ) ) ;
#20369=CARTESIAN_POINT ( 'NONE',  ( -10.60000000000000142, 12.50000000000000000, 0.4115034346978110880 ) ) ;
#20370=FACE_OUTER_BOUND ( 'NONE', #110545, .T. ) ;
#20371=ORIENTED_EDGE ( 'NONE', *, *, #89059, .T. ) ;
#20372=AXIS2_PLACEMENT_3D ( 'NONE', #67049, #48091, #96514 ) ;
#20373=CONICAL_SURFACE ( 'NONE', #116500, 0.1000000000000002554, 0.003490658503988666988 ) ;
#20374=ORIENTED_EDGE ( 'NONE', *, *, #127743, .T. ) ;
#20375=DIRECTION ( 'NONE',  ( -0.000000000000000000, 1.000000000000000000, -0.000000000000000000 ) ) ;
#20376=AXIS2_PLACEMENT_3D ( 'NONE', #15782, #123798, #73417 ) ;
#20377=EDGE_LOOP ( 'NONE', ( #104530, #14664, #654, #79397 ) ) ;
#20379=EDGE_LOOP ( 'NONE', ( #30717, #10619, #122244, #60600 ) ) ;
#20380=ADVANCED_FACE ( 'NONE', ( #7585 ), #90691, .T. ) ;
#20381=ORIENTED_EDGE ( 'NONE', *, *, #123733, .T. ) ;
#20382=CARTESIAN_POINT ( 'NONE',  ( 4.399999999999939071, 12.50000000000000000, 0.3464101615137736845 ) ) ;
#20383=DIRECTION ( 'NONE',  ( 0.000000000000000000, -0.9999939076577903929, 0.003490651415223739937 ) ) ;
#20384=VECTOR ( 'NONE', #30474, 1000.000000000000000 ) ;
#20385=CARTESIAN_POINT ( 'NONE',  ( -13.09999999999999076, 2.500000000000000000, 4.576537180435972019 ) ) ;
#20386=CARTESIAN_POINT ( 'NONE',  ( -2.050000000000032685, 2.500000000000000000, -6.395190528383301931 ) ) ;
#20387=AXIS2_PLACEMENT_3D ( 'NONE', #41601, #2950, #12108 ) ;
#20388=CARTESIAN_POINT ( 'NONE',  ( 87.50000000000001421, 1.433398978532515633, 7.395196794792773254 ) ) ;
#20389=ORIENTED_EDGE ( 'NONE', *, *, #36423, .F. ) ;
#20390=CARTESIAN_POINT ( 'NONE',  ( -1.050000000000038680, 2.500000000000000000, 2.411473670974873862 ) ) ;
#20391=CARTESIAN_POINT ( 'NONE',  ( 11.24999999999990941, 2.500000000000000000, -1.472243186433550122 ) ) ;
#20392=DIRECTION ( 'NONE',  ( 0.000000000000000000, -0.000000000000000000, 1.000000000000000000 ) ) ;
#20393=CARTESIAN_POINT ( 'NONE',  ( 6.899999999999928413, 12.50000000000000000, -3.983716857408426293 ) ) ;
#20394=AXIS2_PLACEMENT_3D ( 'NONE', #64435, #71853, #60739 ) ;
#20395=VECTOR ( 'NONE', #121734, 1000.000000000000000 ) ;
#20396=CARTESIAN_POINT ( 'NONE',  ( -10.65000000000000391, 12.50000000000000000, -6.841600689897075149 ) ) ;
#20397=VERTEX_POINT ( 'NONE', #46229 ) ;
#20398=AXIS2_PLACEMENT_3D ( 'NONE', #4271, #35068, #94598 ) ;
#20399=ADVANCED_FACE ( 'NONE', ( #85512 ), #57246, .T. ) ;
#20400=EDGE_LOOP ( 'NONE', ( #86900, #35127 ) ) ;
#20401=DIRECTION ( 'NONE',  ( 0.000000000000000000, -0.9999939076577903929, 0.003490651415223739937 ) ) ;
#20402=AXIS2_PLACEMENT_3D ( 'NONE', #44135, #72959, #83430 ) ;
#20403=ORIENTED_EDGE ( 'NONE', *, *, #1919, .T. ) ;
#20404=CARTESIAN_POINT ( 'NONE',  ( 3.299999999999942979, 2.500000000000000000, 4.330127018922196314 ) ) ;
#20405=CARTESIAN_POINT ( 'NONE',  ( -14.14999999999998614, 12.50000000000000000, -2.857883832488651521 ) ) ;
#20406=VECTOR ( 'NONE', #5862, 1000.000000000000000 ) ;
#20407=VECTOR ( 'NONE', #42650, 1000.000000000000000 ) ;
#20408=ORIENTED_EDGE ( 'NONE', *, *, #65946, .F. ) ;
#20409=DIRECTION ( 'NONE',  ( 0.000000000000000000, 0.000000000000000000, 1.000000000000000000 ) ) ;
#20410=DIRECTION ( 'NONE',  ( -0.000000000000000000, 1.000000000000000000, -0.000000000000000000 ) ) ;
#20411=VECTOR ( 'NONE', #83619, 1000.000000000000000 ) ;
#20412=ADVANCED_FACE ( 'NONE', ( #6282 ), #126197, .T. ) ;
#20413=CARTESIAN_POINT ( 'NONE',  ( -0.8500000000000390576, 2.500000000000000000, -6.595190528383302109 ) ) ;
#20414=LINE ( 'NONE', #19088, #56025 ) ;
#20415=CIRCLE ( 'NONE', #122919, 0.09999999999999982514 ) ;
#20416=CONICAL_SURFACE ( 'NONE', #37150, 0.09999999999999982514, 0.003490658503988666988 ) ;
#20417=PLANE ( 'NONE',  #54030 ) ;
#20418=ORIENTED_EDGE ( 'NONE', *, *, #161, .T. ) ;
#20419=CARTESIAN_POINT ( 'NONE',  ( 26.76313892655710447, 1.072173145595670452, -4.440523166430129010 ) ) ;
#20420=CARTESIAN_POINT ( 'NONE',  ( 6.899999999999928413, 2.500000000000000000, 3.983716857408420964 ) ) ;
#20421=PLANE ( 'NONE',  #67873 ) ;
#20422=DIRECTION ( 'NONE',  ( -0.000000000000000000, 1.000000000000000000, -0.000000000000000000 ) ) ;
#20423=ORIENTED_EDGE ( 'NONE', *, *, #53522, .F. ) ;
#20424=VERTEX_POINT ( 'NONE', #107733 ) ;
#20425=DIRECTION ( 'NONE',  ( -0.000000000000000000, -1.000000000000000000, -0.000000000000000000 ) ) ;
#20426=CARTESIAN_POINT ( 'NONE',  ( -5.800000000000018474, 12.50000000000000000, 4.330127018922196314 ) ) ;
#20427=AXIS2_PLACEMENT_3D ( 'NONE', #47685, #69232, #97413 ) ;
#20428=DIRECTION ( 'NONE',  ( 0.000000000000000000, 1.000000000000000000, 0.000000000000000000 ) ) ;
#20429=EDGE_LOOP ( 'NONE', ( #117416, #18691 ) ) ;
#20430=DIRECTION ( 'NONE',  ( 0.000000000000000000, -0.9999939076577903929, 0.003490651415223739937 ) ) ;
#20431=EDGE_CURVE ( 'NONE', #71600, #112569, #76022, .T. ) ;
#20432=CARTESIAN_POINT ( 'NONE',  ( -12.69999999999999218, 12.50000000000000000, 4.611443907251934426 ) ) ;
#20433=EDGE_LOOP ( 'NONE', ( #119095, #127340 ) ) ;
#20434=DIRECTION ( 'NONE',  ( 0.000000000000000000, 0.000000000000000000, -1.000000000000000000 ) ) ;
#20435=ORIENTED_EDGE ( 'NONE', *, *, #115865, .T. ) ;
#20436=DIRECTION ( 'NONE',  ( 0.000000000000000000, 0.000000000000000000, 1.000000000000000000 ) ) ;
#20437=EDGE_CURVE ( 'NONE', #33882, #111424, #19592, .T. ) ;
#20438=CONICAL_SURFACE ( 'NONE', #110233, 0.1000000000000002554, 0.003490658503988666988 ) ;
#20439=CIRCLE ( 'NONE', #22614, 0.06509327318403745899 ) ;
#20440=ORIENTED_EDGE ( 'NONE', *, *, #43289, .T. ) ;
#20441=CARTESIAN_POINT ( 'NONE',  ( 9.549999999999918998, 2.500000000000000000, -6.495190528383302464 ) ) ;
#20442=CARTESIAN_POINT ( 'NONE',  ( 15.83209681635555022, 2.500000000000000000, -5.404881881984143099 ) ) ;
#20443=EDGE_CURVE ( 'NONE', #52720, #39660, #99004, .T. ) ;
#20444=VERTEX_POINT ( 'NONE', #59952 ) ;
#20445=EDGE_CURVE ( 'NONE', #60383, #16549, #61468, .T. ) ;
#20446=ORIENTED_EDGE ( 'NONE', *, *, #68139, .F. ) ;
#20447=EDGE_CURVE ( 'NONE', #46996, #17873, #76945, .T. ) ;
#20448=EDGE_CURVE ( 'NONE', #1478, #37337, #34278, .T. ) ;
#20449=CARTESIAN_POINT ( 'NONE',  ( 10.79999999999991012, 2.500000000000000000, -4.330127018922201643 ) ) ;
#20450=DIRECTION ( 'NONE',  ( 0.000000000000000000, 0.000000000000000000, 1.000000000000000000 ) ) ;
#20451=ORIENTED_EDGE ( 'NONE', *, *, #67621, .T. ) ;
#20452=VECTOR ( 'NONE', #41945, 1000.000000000000000 ) ;
#20453=DIRECTION ( 'NONE',  ( 0.000000000000000000, 1.000000000000000000, 0.000000000000000000 ) ) ;
#20454=CARTESIAN_POINT ( 'NONE',  ( -11.84999999999999787, 2.500000000000000000, -1.918653347947322008 ) ) ;
#20455=CIRCLE ( 'NONE', #37193, 0.06509327318403745899 ) ;
#20456=EDGE_CURVE ( 'NONE', #5343, #57940, #109673, .T. ) ;
#20457=DIRECTION ( 'NONE',  ( -0.000000000000000000, -1.000000000000000000, -0.000000000000000000 ) ) ;
#20458=ADVANCED_FACE ( 'NONE', ( #48827 ), #40545, .T. ) ;
#20460=DIRECTION ( 'NONE',  ( 0.000000000000000000, 1.000000000000000000, 0.000000000000000000 ) ) ;
#20461=CARTESIAN_POINT ( 'NONE',  ( 12.04999999999990834, 2.500000000000000000, 6.495190528383297135 ) ) ;
#20462=CARTESIAN_POINT ( 'NONE',  ( 10.44999999999991047, 12.50000000000000000, -6.495190528383302464 ) ) ;
#20463=ADVANCED_FACE ( 'NONE', ( #48170 ), #124134, .T. ) ;
#20464=EDGE_CURVE ( 'NONE', #112146, #58918, #113682, .T. ) ;
#20465=AXIS2_PLACEMENT_3D ( 'NONE', #40623, #110614, #60873 ) ;
#20466=ADVANCED_FACE ( 'NONE', ( #50122 ), #90008, .T. ) ;
#20467=EDGE_LOOP ( 'NONE', ( #125083, #56515 ) ) ;
#20468=ORIENTED_EDGE ( 'NONE', *, *, #77017, .F. ) ;
#20469=ORIENTED_EDGE ( 'NONE', *, *, #79962, .T. ) ;
#20470=DIRECTION ( 'NONE',  ( -0.000000000000000000, -1.000000000000000000, -0.000000000000000000 ) ) ;
#20471=DIRECTION ( 'NONE',  ( 0.000000000000000000, 1.000000000000000000, 0.000000000000000000 ) ) ;
#20472=VECTOR ( 'NONE', #10690, 1000.000000000000000 ) ;
#20473=CARTESIAN_POINT ( 'NONE',  ( 4.549999999999935874, 2.500000000000000000, 6.495190528383297135 ) ) ;
#20474=VERTEX_POINT ( 'NONE', #40292 ) ;
#20475=EDGE_LOOP ( 'NONE', ( #63156, #66902, #60846, #66480 ) ) ;
#20476=FACE_BOUND ( 'NONE', #77775, .T. ) ;
#20477=ORIENTED_EDGE ( 'NONE', *, *, #34492, .T. ) ;
#20478=EDGE_CURVE ( 'NONE', #49092, #81291, #9124, .T. ) ;
#20479=CARTESIAN_POINT ( 'NONE',  ( 12.89999999999990266, 2.500000000000000000, 5.122947341949749323 ) ) ;
#20480=DIRECTION ( 'NONE',  ( 0.000000000000000000, 0.000000000000000000, 1.000000000000000000 ) ) ;
#20482=AXIS2_PLACEMENT_3D ( 'NONE', #47008, #65330, #86911 ) ;
#20483=DIRECTION ( 'NONE',  ( -4.274815082592931898E-19, -0.9999939076577903929, -0.003490651415223739937 ) ) ;
#20484=DIRECTION ( 'NONE',  ( 0.000000000000000000, 0.000000000000000000, 1.000000000000000000 ) ) ;
#20485=DIRECTION ( 'NONE',  ( -0.000000000000000000, 1.000000000000000000, -0.000000000000000000 ) ) ;
#20486=AXIS2_PLACEMENT_3D ( 'NONE', #49982, #107590, #38884 ) ;
#20487=DIRECTION ( 'NONE',  ( 0.000000000000000000, -0.000000000000000000, 1.000000000000000000 ) ) ;
#20488=CARTESIAN_POINT ( 'NONE',  ( 15.59999999999988951, 12.50000000000000000, -0.2813168883297409439 ) ) ;
#20489=DIRECTION ( 'NONE',  ( 0.000000000000000000, 1.000000000000000000, 0.000000000000000000 ) ) ;
#20490=AXIS2_PLACEMENT_3D ( 'NONE', #21634, #122419, #12438 ) ;
#20491=DIRECTION ( 'NONE',  ( -0.000000000000000000, 1.000000000000000000, -0.000000000000000000 ) ) ;
#20492=EDGE_LOOP ( 'NONE', ( #58523, #75477 ) ) ;
#20493=CIRCLE ( 'NONE', #64391, 0.1000000000000002554 ) ;
#20494=ORIENTED_EDGE ( 'NONE', *, *, #29650, .F. ) ;
#20495=EDGE_LOOP ( 'NONE', ( #64592, #43412, #30172, #2556 ) ) ;
#20496=ORIENTED_EDGE ( 'NONE', *, *, #128983, .F. ) ;
#20497=DIRECTION ( 'NONE',  ( -0.000000000000000000, 1.000000000000000000, -0.000000000000000000 ) ) ;
#20498=PLANE ( 'NONE',  #111277 ) ;
#20499=VERTEX_POINT ( 'NONE', #78292 ) ;
#20500=ORIENTED_EDGE ( 'NONE', *, *, #121700, .F. ) ;
#20501=AXIS2_PLACEMENT_3D ( 'NONE', #23701, #64260, #41428 ) ;
#20502=VERTEX_POINT ( 'NONE', #78935 ) ;
#20503=CARTESIAN_POINT ( 'NONE',  ( -14.59999999999998366, 2.500000000000000000, -0.6928203230275520319 ) ) ;
#20504=AXIS2_PLACEMENT_3D ( 'NONE', #25135, #54584, #105645 ) ;
#20505=CIRCLE ( 'NONE', #10034, 0.06509327318403741736 ) ;
#20506=DIRECTION ( 'NONE',  ( 0.000000000000000000, 1.000000000000000000, 0.000000000000000000 ) ) ;
#20507=DIRECTION ( 'NONE',  ( 0.000000000000000000, 0.000000000000000000, 1.000000000000000000 ) ) ;
#20508=CARTESIAN_POINT ( 'NONE',  ( -8.950000000000004619, 2.500000000000000000, 6.248780366869521430 ) ) ;
#20509=FACE_OUTER_BOUND ( 'NONE', #54767, .T. ) ;
#20510=DIRECTION ( 'NONE',  ( -4.274815082592931898E-19, -0.9999939076577903929, -0.003490651415223739937 ) ) ;
#20511=CARTESIAN_POINT ( 'NONE',  ( 9.149999999999920419, 12.50000000000000000, -5.802370205355749988 ) ) ;
#20512=AXIS2_PLACEMENT_3D ( 'NONE', #104533, #53513, #86157 ) ;
#20513=ORIENTED_EDGE ( 'NONE', *, *, #8051, .T. ) ;
#20514=FACE_OUTER_BOUND ( 'NONE', #111969, .T. ) ;
#20515=EDGE_LOOP ( 'NONE', ( #48007, #33381 ) ) ;
#20516=EDGE_CURVE ( 'NONE', #111617, #7920, #84432, .T. ) ;
#20517=CIRCLE ( 'NONE', #116638, 0.1000000000000000056 ) ;
#20518=ORIENTED_EDGE ( 'NONE', *, *, #124061, .F. ) ;
#20519=EDGE_LOOP ( 'NONE', ( #5342, #49334, #94913, #3877 ) ) ;
#20520=ADVANCED_FACE ( 'NONE', ( #88737 ), #29721, .T. ) ;
#20522=ORIENTED_EDGE ( 'NONE', *, *, #88298, .F. ) ;
#20523=ORIENTED_EDGE ( 'NONE', *, *, #33352, .F. ) ;
#20524=DIRECTION ( 'NONE',  ( 0.000000000000000000, 1.000000000000000000, 0.000000000000000000 ) ) ;
#20526=DIRECTION ( 'NONE',  ( -0.000000000000000000, 1.000000000000000000, -0.000000000000000000 ) ) ;
#20527=CARTESIAN_POINT ( 'NONE',  ( -2.900000000000029221, 2.500000000000000000, -0.5928203230275541635 ) ) ;
#20528=DIRECTION ( 'NONE',  ( -4.274815082592931898E-19, -0.9999939076577903929, -0.003490651415223739937 ) ) ;
#20529=LINE ( 'NONE', #70269, #103436 ) ;
#20530=CARTESIAN_POINT ( 'NONE',  ( -3.950000000000026379, 2.500000000000000000, 2.511473670974873507 ) ) ;
#20531=DIRECTION ( 'NONE',  ( -4.274815082592931898E-19, -0.9999939076577903929, -0.003490651415223739937 ) ) ;
#20532=ORIENTED_EDGE ( 'NONE', *, *, #77601, .F. ) ;
#20533=DIRECTION ( 'NONE',  ( -0.000000000000000000, 1.000000000000000000, -0.000000000000000000 ) ) ;
#20534=ORIENTED_EDGE ( 'NONE', *, *, #102598, .T. ) ;
#20536=DIRECTION ( 'NONE',  ( -4.274815082592931898E-19, -0.9999939076577903929, -0.003490651415223739937 ) ) ;
#20537=AXIS2_PLACEMENT_3D ( 'NONE', #123654, #32741, #92941 ) ;
#20538=AXIS2_PLACEMENT_3D ( 'NONE', #8415, #47720, #100039 ) ;
#20539=EDGE_LOOP ( 'NONE', ( #22348, #121340 ) ) ;
#20540=DIRECTION ( 'NONE',  ( 0.000000000000000000, -0.9999939076577903929, 0.003490651415223739937 ) ) ;
#20541=AXIS2_PLACEMENT_3D ( 'NONE', #101294, #81005, #120923 ) ;
#20542=CARTESIAN_POINT ( 'NONE',  ( 6.449999999999933564, 2.500000000000000000, -6.841600689897078702 ) ) ;
#20543=EDGE_LOOP ( 'NONE', ( #113646, #64467, #9979, #123617 ) ) ;
#20544=CARTESIAN_POINT ( 'NONE',  ( 6.649999999999931966, 2.500000000000000000, -5.802370205355749988 ) ) ;
#20545=ORIENTED_EDGE ( 'NONE', *, *, #75242, .F. ) ;
#20546=ORIENTED_EDGE ( 'NONE', *, *, #124426, .F. ) ;
#20547=CARTESIAN_POINT ( 'NONE',  ( 9.799999999999915445, 2.500000000000000000, 3.983716857408420964 ) ) ;
#20549=LINE ( 'NONE', #38928, #77301 ) ;
#20550=DIRECTION ( 'NONE',  ( 0.000000000000000000, 1.000000000000000000, 0.000000000000000000 ) ) ;
#20551=AXIS2_PLACEMENT_3D ( 'NONE', #58111, #79046, #69187 ) ;
#20552=DIRECTION ( 'NONE',  ( 0.000000000000000000, 1.000000000000000000, 0.000000000000000000 ) ) ;
#20553=VECTOR ( 'NONE', #121038, 1000.000000000000000 ) ;
#20554=VERTEX_POINT ( 'NONE', #67562 ) ;
#20555=FACE_OUTER_BOUND ( 'NONE', #114658, .T. ) ;
#20556=ORIENTED_EDGE ( 'NONE', *, *, #100842, .F. ) ;
#20557=CARTESIAN_POINT ( 'NONE',  ( 12.89999999999990088, 12.50000000000000000, 4.330127018922196314 ) ) ;
#20558=CARTESIAN_POINT ( 'NONE',  ( 9.349999999999916156, 2.500000000000000000, 6.048780366869520364 ) ) ;
#20559=AXIS2_PLACEMENT_3D ( 'NONE', #95491, #5800, #75838 ) ;
#20560=EDGE_CURVE ( 'NONE', #65002, #65711, #47951, .T. ) ;
#20561=EDGE_CURVE ( 'NONE', #113501, #104378, #44386, .T. ) ;
#20562=AXIS2_PLACEMENT_3D ( 'NONE', #25685, #55799, #83342 ) ;
#20564=CARTESIAN_POINT ( 'NONE',  ( 0.8499999999999553468, 2.500000000000000000, 1.472243186433545459 ) ) ;
#20565=DIRECTION ( 'NONE',  ( 0.000000000000000000, 0.000000000000000000, 1.000000000000000000 ) ) ;
#20566=EDGE_CURVE ( 'NONE', #85870, #101480, #61115, .T. ) ;
#20567=DIRECTION ( 'NONE',  ( -0.000000000000000000, -1.000000000000000000, -0.000000000000000000 ) ) ;
#20568=CARTESIAN_POINT ( 'NONE',  ( -1.900000000000034106, 12.50000000000000000, -3.983716857408426293 ) ) ;
#20569=VERTEX_POINT ( 'NONE', #5427 ) ;
#20570=CIRCLE ( 'NONE', #104186, 0.06509327318403745899 ) ;
#20571=CARTESIAN_POINT ( 'NONE',  ( 6.249999999999967137, 12.50000000000000000, -2.165063509461101710 ) ) ;
#20572=CARTESIAN_POINT ( 'NONE',  ( -2.700000000000029932, 2.500000000000000000, -4.676537180435977881 ) ) ;
#20573=DIRECTION ( 'NONE',  ( 0.000000000000000000, 0.000000000000000000, 1.000000000000000000 ) ) ;
#20575=ADVANCED_FACE ( 'NONE', ( #26379 ), #2509, .T. ) ;
#20576=ORIENTED_EDGE ( 'NONE', *, *, #88592, .T. ) ;
#20577=CIRCLE ( 'NONE', #31060, 0.06509327318403745899 ) ;
#20578=CARTESIAN_POINT ( 'NONE',  ( -9.150000000000009237, 12.50000000000000000, -7.188010851410848723 ) ) ;
#20579=VECTOR ( 'NONE', #49891, 1000.000000000000000 ) ;
#20581=ORIENTED_EDGE ( 'NONE', *, *, #47067, .F. ) ;
#20582=FACE_OUTER_BOUND ( 'NONE', #88489, .T. ) ;
#20583=EDGE_LOOP ( 'NONE', ( #21812, #16321 ) ) ;
#20584=AXIS2_PLACEMENT_3D ( 'NONE', #114014, #91789, #43349 ) ;
#20585=DIRECTION ( 'NONE',  ( 0.000000000000000000, 0.000000000000000000, 1.000000000000000000 ) ) ;
#20586=DIRECTION ( 'NONE',  ( 0.000000000000000000, 0.000000000000000000, 1.000000000000000000 ) ) ;
#20587=ORIENTED_EDGE ( 'NONE', *, *, #9466, .T. ) ;
#20588=FACE_OUTER_BOUND ( 'NONE', #67524, .T. ) ;
#20590=CARTESIAN_POINT ( 'NONE',  ( -5.400000000000024336, 12.50000000000000000, -3.702399969078687292 ) ) ;
#20591=FACE_OUTER_BOUND ( 'NONE', #66634, .T. ) ;
#20592=AXIS2_PLACEMENT_3D ( 'NONE', #38507, #9009, #36572 ) ;
#20593=ORIENTED_EDGE ( 'NONE', *, *, #117412, .T. ) ;
#20594=EDGE_CURVE ( 'NONE', #82955, #9027, #104911, .T. ) ;
#20595=CONICAL_SURFACE ( 'NONE', #110472, 0.1000000000000002554, 0.003490658503988666988 ) ;
#20596=CIRCLE ( 'NONE', #81240, 0.06509327318403745899 ) ;
#20597=VERTEX_POINT ( 'NONE', #97043 ) ;
#20598=EDGE_LOOP ( 'NONE', ( #96980, #107622, #105929, #25230 ) ) ;
#20599=CARTESIAN_POINT ( 'NONE',  ( 1.449999999999949551, 12.50000000000000000, 6.841600689897072485 ) ) ;
#20600=CARTESIAN_POINT ( 'NONE',  ( -3.950000000000026379, 12.50000000000000000, 6.906693963081109722 ) ) ;
#20601=CARTESIAN_POINT ( 'NONE',  ( 17.50000000000000000, -2.500000000000000000, -3.999999999999998224 ) ) ;
#20602=EDGE_CURVE ( 'NONE', #93533, #100605, #86127, .T. ) ;
#20603=EDGE_CURVE ( 'NONE', #18475, #76431, #31787, .T. ) ;
#20604=FACE_BOUND ( 'NONE', #35246, .T. ) ;
#20605=ORIENTED_EDGE ( 'NONE', *, *, #13034, .F. ) ;
#20606=ADVANCED_FACE ( 'NONE', ( #37494 ), #96379, .T. ) ;
#20607=ADVANCED_FACE ( 'NONE', ( #117287 ), #121654, .T. ) ;
#20608=DIRECTION ( 'NONE',  ( -0.000000000000000000, 1.000000000000000000, -0.000000000000000000 ) ) ;
#20609=PLANE ( 'NONE',  #27202 ) ;
#20610=ORIENTED_EDGE ( 'NONE', *, *, #122019, .F. ) ;
#20611=DIRECTION ( 'NONE',  ( 0.000000000000000000, 1.000000000000000000, 0.000000000000000000 ) ) ;
#20612=CARTESIAN_POINT ( 'NONE',  ( 17.02136413300363316, 1.939324994459781903, 5.540650668389440980 ) ) ;
#20613=EDGE_CURVE ( 'NONE', #53623, #66905, #6694, .T. ) ;
#20614=LINE ( 'NONE', #80174, #96687 ) ;
#20615=DIRECTION ( 'NONE',  ( 0.000000000000000000, 1.000000000000000000, 0.000000000000000000 ) ) ;
#20616=AXIS2_PLACEMENT_3D ( 'NONE', #100923, #80006, #91119 ) ;
#20617=DIRECTION ( 'NONE',  ( 0.000000000000000000, 0.000000000000000000, -1.000000000000000000 ) ) ;
#20618=EDGE_CURVE ( 'NONE', #41193, #49661, #65204, .T. ) ;
#20619=FACE_OUTER_BOUND ( 'NONE', #120932, .T. ) ;
#20620=DIRECTION ( 'NONE',  ( -0.000000000000000000, 1.000000000000000000, -0.000000000000000000 ) ) ;
#20621=EDGE_CURVE ( 'NONE', #104101, #114153, #15023, .T. ) ;
#20622=VECTOR ( 'NONE', #59701, 1000.000000000000000 ) ;
#20623=ADVANCED_FACE ( 'NONE', ( #15892 ), #68215, .T. ) ;
#20624=ORIENTED_EDGE ( 'NONE', *, *, #102174, .F. ) ;
#20625=ORIENTED_EDGE ( 'NONE', *, *, #20448, .F. ) ;
#20626=AXIS2_PLACEMENT_3D ( 'NONE', #22142, #20834, #122902 ) ;
#20627=VERTEX_POINT ( 'NONE', #35558 ) ;
#20628=VERTEX_POINT ( 'NONE', #75459 ) ;
#20629=FACE_OUTER_BOUND ( 'NONE', #18352, .T. ) ;
#20630=CARTESIAN_POINT ( 'NONE',  ( -14.59999999999998366, 12.50000000000000000, 0.6928203230275518099 ) ) ;
#20631=EDGE_LOOP ( 'NONE', ( #31312, #81571 ) ) ;
#20632=EDGE_CURVE ( 'NONE', #105063, #34708, #85913, .T. ) ;
#20633=FACE_BOUND ( 'NONE', #21271, .T. ) ;
#20634=EDGE_CURVE ( 'NONE', #64406, #55074, #90339, .T. ) ;
#20635=LINE ( 'NONE', #10769, #87566 ) ;
#20636=CONICAL_SURFACE ( 'NONE', #93790, 0.1000000000000002554, 0.003490658503988666988 ) ;
#20637=CARTESIAN_POINT ( 'NONE',  ( 16.55874544816223448, 0.4845305829267578801, 6.091953208799004926 ) ) ;
#20638=CONICAL_SURFACE ( 'NONE', #22799, 0.09999999999999982514, 0.003490658503988666988 ) ;
#20639=AXIS2_PLACEMENT_3D ( 'NONE', #1470, #23058, #91155 ) ;
#20640=CARTESIAN_POINT ( 'NONE',  ( -2.300000000000032685, 2.500000000000000000, -0.3464101615137783474 ) ) ;
#20641=DIRECTION ( 'NONE',  ( 0.000000000000000000, 0.000000000000000000, 1.000000000000000000 ) ) ;
#20642=CARTESIAN_POINT ( 'NONE',  ( -11.44999999999999929, 12.50000000000000000, -1.818653347947322141 ) ) ;
#20643=CARTESIAN_POINT ( 'NONE',  ( -4.600000000000024514, 2.500000000000000000, 4.922947341949748257 ) ) ;
#20644=CARTESIAN_POINT ( 'NONE',  ( -5.200000000000022382, 12.50000000000000000, 4.611443907251934426 ) ) ;
#20645=DIRECTION ( 'NONE',  ( 0.000000000000000000, 0.000000000000000000, 1.000000000000000000 ) ) ;
#20646=EDGE_LOOP ( 'NONE', ( #65292, #31151, #63012, #73116 ) ) ;
#20647=CIRCLE ( 'NONE', #1844, 0.06509327318403745899 ) ;
#20648=ORIENTED_EDGE ( 'NONE', *, *, #18720, .T. ) ;
#20649=AXIS2_PLACEMENT_3D ( 'NONE', #92996, #43260, #21016 ) ;
#20650=ORIENTED_EDGE ( 'NONE', *, *, #1246, .T. ) ;
#20651=ORIENTED_EDGE ( 'NONE', *, *, #127596, .T. ) ;
#20652=EDGE_LOOP ( 'NONE', ( #40408, #82359, #17756, #17668 ) ) ;
#20653=EDGE_LOOP ( 'NONE', ( #25752, #79476, #100638, #68023 ) ) ;
#20654=CARTESIAN_POINT ( 'NONE',  ( 3.949999999999941558, 2.500000000000000000, -6.148780366869526226 ) ) ;
#20655=ORIENTED_EDGE ( 'NONE', *, *, #32292, .F. ) ;
#20656=AXIS2_PLACEMENT_3D ( 'NONE', #34997, #85357, #15306 ) ;
#20657=CARTESIAN_POINT ( 'NONE',  ( 10.84999999999990905, 12.50000000000000000, 2.099970236277060032 ) ) ;
#20659=LINE ( 'NONE', #61223, #91771 ) ;
#20660=CARTESIAN_POINT ( 'NONE',  ( 1.249999999999988898, 2.500000000000000000, -6.595190528383302109 ) ) ;
#20661=AXIS2_PLACEMENT_3D ( 'NONE', #80603, #50486, #100241 ) ;
#20662=ORIENTED_EDGE ( 'NONE', *, *, #85436, .T. ) ;
#20663=CARTESIAN_POINT ( 'NONE',  ( -8.150000000000012790, 12.50000000000000000, 1.818653347947321475 ) ) ;
#20664=VERTEX_POINT ( 'NONE', #30899 ) ;
#20665=EDGE_CURVE ( 'NONE', #96497, #24701, #8772, .T. ) ;
#20666=VERTEX_POINT ( 'NONE', #765 ) ;
#20667=CONICAL_SURFACE ( 'NONE', #68768, 0.1000000000000002554, 0.003490658503988666988 ) ;
#20668=CARTESIAN_POINT ( 'NONE',  ( -7.499999999999976907, 2.500000000000000000, 4.330127018922196314 ) ) ;
#20669=EDGE_CURVE ( 'NONE', #92919, #117157, #1408, .T. ) ;
#20670=FACE_OUTER_BOUND ( 'NONE', #129, .T. ) ;
#20671=CARTESIAN_POINT ( 'NONE',  ( 10.39999999999990976, 12.50000000000000000, 4.330127018922196314 ) ) ;
#20672=ORIENTED_EDGE ( 'NONE', *, *, #71394, .T. ) ;
#20673=VECTOR ( 'NONE', #67669, 1000.000000000000000 ) ;
#20674=VERTEX_POINT ( 'NONE', #59057 ) ;
#20675=DIRECTION ( 'NONE',  ( 0.000000000000000000, 1.000000000000000000, 0.000000000000000000 ) ) ;
#20676=AXIS2_PLACEMENT_3D ( 'NONE', #15729, #15061, #25542 ) ;
#20677=LINE ( 'NONE', #109025, #95542 ) ;
#20678=DIRECTION ( 'NONE',  ( 0.000000000000000000, 1.000000000000000000, 0.000000000000000000 ) ) ;
#20679=LINE ( 'NONE', #22626, #35709 ) ;
#20680=VERTEX_POINT ( 'NONE', #40059 ) ;
#20681=CARTESIAN_POINT ( 'NONE',  ( 0.5999999999999612310, 2.500000000000000000, -0.2464101615137760659 ) ) ;
#20682=AXIS2_PLACEMENT_3D ( 'NONE', #85368, #125297, #35635 ) ;
#20683=ORIENTED_EDGE ( 'NONE', *, *, #43832, .F. ) ;
#20684=CARTESIAN_POINT ( 'NONE',  ( 10.84999999999991260, 2.500000000000000000, 5.802370205355744659 ) ) ;
#20685=ORIENTED_EDGE ( 'NONE', *, *, #65368, .T. ) ;
#20686=DIRECTION ( 'NONE',  ( 0.000000000000000000, 0.000000000000000000, -1.000000000000000000 ) ) ;
#20687=AXIS2_PLACEMENT_3D ( 'NONE', #50488, #39412, #19755 ) ;
#20688=CARTESIAN_POINT ( 'NONE',  ( -11.44999999999999751, 12.50000000000000000, -2.511473670974873951 ) ) ;
#20690=AXIS2_PLACEMENT_3D ( 'NONE', #51541, #101919, #79691 ) ;
#20691=CARTESIAN_POINT ( 'NONE',  ( 12.94999999999989981, 12.50000000000000000, -2.165063509461101710 ) ) ;
#20692=VERTEX_POINT ( 'NONE', #81274 ) ;
#20693=CARTESIAN_POINT ( 'NONE',  ( 6.649999999999930189, 2.500000000000000000, -1.472243186433550122 ) ) ;
#20694=AXIS2_PLACEMENT_3D ( 'NONE', #22164, #52250, #92159 ) ;
#20695=VECTOR ( 'NONE', #49566, 1000.000000000000000 ) ;
#20696=DIRECTION ( 'NONE',  ( 0.000000000000000000, 0.000000000000000000, 1.000000000000000000 ) ) ;
#20697=VERTEX_POINT ( 'NONE', #58423 ) ;
#20698=ORIENTED_EDGE ( 'NONE', *, *, #55096, .T. ) ;
#20699=VERTEX_POINT ( 'NONE', #98975 ) ;
#20700=CARTESIAN_POINT ( 'NONE',  ( -1.050000000000037348, 2.500000000000000000, -6.941600689897078347 ) ) ;
#20701=DIRECTION ( 'NONE',  ( 0.000000000000000000, 0.000000000000000000, 1.000000000000000000 ) ) ;
#20702=FACE_OUTER_BOUND ( 'NONE', #60303, .T. ) ;
#20703=CARTESIAN_POINT ( 'NONE',  ( 4.399999999999939071, 2.500000000000000000, -0.4464101615137782142 ) ) ;
#20704=CARTESIAN_POINT ( 'NONE',  ( -7.100000000000018296, 2.500000000000000000, -2.385244779468109755E-15 ) ) ;
#20705=ADVANCED_FACE ( 'NONE', ( #28960 ), #25502, .T. ) ;
#20706=DIRECTION ( 'NONE',  ( 0.000000000000000000, 0.000000000000000000, -1.000000000000000000 ) ) ;
#20707=CARTESIAN_POINT ( 'NONE',  ( 0.8499999999999557909, 12.50000000000000000, -6.495190528383302464 ) ) ;
#20708=DIRECTION ( 'NONE',  ( 0.000000000000000000, -0.000000000000000000, 1.000000000000000000 ) ) ;
#20709=CIRCLE ( 'NONE', #123109, 0.06509327318403745899 ) ;
#20710=AXIS2_PLACEMENT_3D ( 'NONE', #18928, #49717, #40546 ) ;
#20711=CIRCLE ( 'NONE', #37448, 0.06509327318403745899 ) ;
#20712=EDGE_LOOP ( 'NONE', ( #72475, #110483, #14939, #58853 ) ) ;
#20713=CARTESIAN_POINT ( 'NONE',  ( -7.900000000000014566, 2.500000000000000000, 0.6928203230275494784 ) ) ;
#20714=ADVANCED_FACE ( 'NONE', ( #69498 ), #18476, .T. ) ;
#20715=DIRECTION ( 'NONE',  ( -4.274815082592931898E-19, -0.9999939076577903929, -0.003490651415223739937 ) ) ;
#20716=ADVANCED_FACE ( 'NONE', ( #108143 ), #8635, .T. ) ;
#20717=DIRECTION ( 'NONE',  ( 0.000000000000000000, -0.9999939076577903929, 0.003490651415223739937 ) ) ;
#20718=DIRECTION ( 'NONE',  ( 0.000000000000000000, -0.000000000000000000, 1.000000000000000000 ) ) ;
#20719=AXIS2_PLACEMENT_3D ( 'NONE', #26509, #87334, #97172 ) ;
#20720=ORIENTED_EDGE ( 'NONE', *, *, #29630, .F. ) ;
#20721=AXIS2_PLACEMENT_3D ( 'NONE', #59507, #19546, #31324 ) ;
#20722=CARTESIAN_POINT ( 'NONE',  ( -3.150000000000029221, 2.500000000000000000, -1.818653347947326138 ) ) ;
#20723=VECTOR ( 'NONE', #119824, 1000.000000000000000 ) ;
#20724=CARTESIAN_POINT ( 'NONE',  ( -5.400000000000024336, 12.50000000000000000, -3.637306695894650055 ) ) ;
#20725=DIRECTION ( 'NONE',  ( 0.000000000000000000, 0.000000000000000000, 1.000000000000000000 ) ) ;
#20726=EDGE_LOOP ( 'NONE', ( #125158, #99235, #85175, #44838 ) ) ;
#20727=ADVANCED_FACE ( 'NONE', ( #11224 ), #55914, .T. ) ;
#20728=AXIS2_PLACEMENT_3D ( 'NONE', #14615, #53294, #84668 ) ;
#20729=ORIENTED_EDGE ( 'NONE', *, *, #72016, .T. ) ;
#20730=DIRECTION ( 'NONE',  ( 0.000000000000000000, -0.9999939076577903929, 0.003490651415223739937 ) ) ;
#20731=AXIS2_PLACEMENT_3D ( 'NONE', #72561, #92175, #31350 ) ;
#20732=ORIENTED_EDGE ( 'NONE', *, *, #117314, .F. ) ;
#20733=ORIENTED_EDGE ( 'NONE', *, *, #80608, .F. ) ;
#20734=FACE_OUTER_BOUND ( 'NONE', #118773, .T. ) ;
#20735=CARTESIAN_POINT ( 'NONE',  ( 21.15177371151439090, 2.593223176056364210, -4.151029080743463773 ) ) ;
#20736=CARTESIAN_POINT ( 'NONE',  ( -7.950000000000012612, 12.50000000000000000, -2.230156782645139391 ) ) ;
#20737=FACE_OUTER_BOUND ( 'NONE', #24058, .T. ) ;
#20738=EDGE_LOOP ( 'NONE', ( #89083, #125224, #110788, #58151 ) ) ;
#20739=DIRECTION ( 'NONE',  ( -0.000000000000000000, -1.000000000000000000, -0.000000000000000000 ) ) ;
#20740=ORIENTED_EDGE ( 'NONE', *, *, #88120, .T. ) ;
#20741=VECTOR ( 'NONE', #120206, 1000.000000000000000 ) ;
#20742=LINE ( 'NONE', #30582, #95577 ) ;
#20744=CARTESIAN_POINT ( 'NONE',  ( 16.80072262464533139, -1.717570462274074838, 5.816823748342618394 ) ) ;
#20745=ORIENTED_EDGE ( 'NONE', *, *, #46690, .T. ) ;
#20746=EDGE_CURVE ( 'NONE', #17252, #95053, #39348, .T. ) ;
#20747=ORIENTED_EDGE ( 'NONE', *, *, #87828, .F. ) ;
#20748=ORIENTED_EDGE ( 'NONE', *, *, #121508, .F. ) ;
#20749=ORIENTED_EDGE ( 'NONE', *, *, #2884, .T. ) ;
#20750=FACE_OUTER_BOUND ( 'NONE', #104807, .T. ) ;
#20751=CARTESIAN_POINT ( 'NONE',  ( 16.04744069018201458, 1.499999999999809042, 6.586254744912538150 ) ) ;
#20752=CARTESIAN_POINT ( 'NONE',  ( -11.24999999999996270, 12.50000000000000000, 6.430097255199259010 ) ) ;
#20753=EDGE_CURVE ( 'NONE', #106287, #18828, #81936, .T. ) ;
#20754=FACE_BOUND ( 'NONE', #86902, .T. ) ;
#20755=CARTESIAN_POINT ( 'NONE',  ( 7.499999999999927169, 2.500000000000000000, -5.122947341949753763 ) ) ;
#20756=FACE_OUTER_BOUND ( 'NONE', #10595, .T. ) ;
#20757=AXIS2_PLACEMENT_3D ( 'NONE', #60468, #80084, #118713 ) ;
#20758=EDGE_CURVE ( 'NONE', #63832, #87480, #98875, .T. ) ;
#20759=LINE ( 'NONE', #12213, #101257 ) ;
#20760=DIRECTION ( 'NONE',  ( 0.000000000000000000, 0.000000000000000000, -1.000000000000000000 ) ) ;
#20762=DIRECTION ( 'NONE',  ( 0.000000000000000000, 1.000000000000000000, 0.000000000000000000 ) ) ;
#20763=EDGE_CURVE ( 'NONE', #101014, #51535, #48494, .T. ) ;
#20764=CARTESIAN_POINT ( 'NONE',  ( -11.44999999999999751, 12.50000000000000000, 6.148780366869520897 ) ) ;
#20765=AXIS2_PLACEMENT_3D ( 'NONE', #16611, #106926, #57857 ) ;
#20766=EDGE_CURVE ( 'NONE', #112120, #114810, #42253, .T. ) ;
#20767=DIRECTION ( 'NONE',  ( -0.000000000000000000, 1.000000000000000000, -0.000000000000000000 ) ) ;
#20768=EDGE_CURVE ( 'NONE', #42757, #103996, #58975, .T. ) ;
#20769=DIRECTION ( 'NONE',  ( 0.000000000000000000, 1.000000000000000000, 0.000000000000000000 ) ) ;
#20770=AXIS2_PLACEMENT_3D ( 'NONE', #405, #12802, #39738 ) ;
#20771=AXIS2_PLACEMENT_3D ( 'NONE', #107196, #77725, #16221 ) ;
#20772=EDGE_CURVE ( 'NONE', #32556, #108826, #119165, .T. ) ;
#20773=VERTEX_POINT ( 'NONE', #29504 ) ;
#20774=ORIENTED_EDGE ( 'NONE', *, *, #83446, .F. ) ;
#20775=EDGE_LOOP ( 'NONE', ( #75398, #35275 ) ) ;
#20776=EDGE_LOOP ( 'NONE', ( #54107, #91308 ) ) ;
#20777=DIRECTION ( 'NONE',  ( 0.000000000000000000, 1.000000000000000000, 0.000000000000000000 ) ) ;
#20778=AXIS2_PLACEMENT_3D ( 'NONE', #66490, #16725, #56658 ) ;
#20779=CARTESIAN_POINT ( 'NONE',  ( -5.800000000000022027, 12.50000000000000000, -4.330127018922201643 ) ) ;
#20780=VERTEX_POINT ( 'NONE', #69410 ) ;
#20781=FACE_BOUND ( 'NONE', #116104, .T. ) ;
#20782=EDGE_CURVE ( 'NONE', #16737, #11179, #38130, .T. ) ;
#20783=FACE_OUTER_BOUND ( 'NONE', #13952, .T. ) ;
#20784=AXIS2_PLACEMENT_3D ( 'NONE', #47587, #78343, #46951 ) ;
#20785=CIRCLE ( 'NONE', #64595, 0.1000000000000000472 ) ;
#20786=EDGE_LOOP ( 'NONE', ( #1151, #6783, #114498, #42864 ) ) ;
#20787=FACE_OUTER_BOUND ( 'NONE', #110259, .T. ) ;
#20788=CARTESIAN_POINT ( 'NONE',  ( 4.549999999999939426, 2.500000000000000000, -6.595190528383302109 ) ) ;
#20789=LINE ( 'NONE', #49619, #124219 ) ;
#20790=FACE_OUTER_BOUND ( 'NONE', #49300, .T. ) ;
#20791=ORIENTED_EDGE ( 'NONE', *, *, #17921, .F. ) ;
#20792=DIRECTION ( 'NONE',  ( 0.000000000000000000, 0.000000000000000000, 1.000000000000000000 ) ) ;
#20793=EDGE_LOOP ( 'NONE', ( #66660, #14510 ) ) ;
#20794=EDGE_LOOP ( 'NONE', ( #38465, #44854 ) ) ;
#20795=CONICAL_SURFACE ( 'NONE', #129487, 0.1000000000000002554, 0.003490658503988666988 ) ;
#20796=DIRECTION ( 'NONE',  ( 0.000000000000000000, 0.000000000000000000, -1.000000000000000000 ) ) ;
#20797=CARTESIAN_POINT ( 'NONE',  ( 14.39999999999989555, 2.500000000000000000, 0.4464101615137736623 ) ) ;
#20798=VERTEX_POINT ( 'NONE', #9862 ) ;
#20799=CARTESIAN_POINT ( 'NONE',  ( 9.349999999999919709, 2.500000000000000000, -6.941600689897078347 ) ) ;
#20800=AXIS2_PLACEMENT_3D ( 'NONE', #66595, #44380, #126166 ) ;
#20801=DIRECTION ( 'NONE',  ( -0.000000000000000000, -1.000000000000000000, -0.000000000000000000 ) ) ;
#20803=DIRECTION ( 'NONE',  ( 0.000000000000000000, 0.000000000000000000, 1.000000000000000000 ) ) ;
#20804=DIRECTION ( 'NONE',  ( 0.000000000000000000, 0.000000000000000000, 1.000000000000000000 ) ) ;
#20805=ORIENTED_EDGE ( 'NONE', *, *, #2418, .T. ) ;
#20806=DIRECTION ( 'NONE',  ( 0.000000000000000000, 0.000000000000000000, 1.000000000000000000 ) ) ;
#20807=AXIS2_PLACEMENT_3D ( 'NONE', #46622, #47286, #105556 ) ;
#20808=ORIENTED_EDGE ( 'NONE', *, *, #111801, .F. ) ;
#20809=CARTESIAN_POINT ( 'NONE',  ( -3.300000000000027800, 2.500000000000000000, -2.276824562219559311E-15 ) ) ;
#20810=AXIS2_PLACEMENT_3D ( 'NONE', #110975, #50791, #52088 ) ;
#20811=CIRCLE ( 'NONE', #81453, 0.1000000000000002554 ) ;
#20812=ORIENTED_EDGE ( 'NONE', *, *, #67084, .F. ) ;
#20813=ADVANCED_FACE ( 'NONE', ( #49802 ), #52704, .T. ) ;
#20815=ORIENTED_EDGE ( 'NONE', *, *, #1538, .F. ) ;
#20816=CARTESIAN_POINT ( 'NONE',  ( -10.60000000000000142, 2.500000000000000000, -0.3464101615137782364 ) ) ;
#20817=LINE ( 'NONE', #30000, #6887 ) ;
#20818=DIRECTION ( 'NONE',  ( 0.000000000000000000, 0.000000000000000000, 1.000000000000000000 ) ) ;
#20819=DIRECTION ( 'NONE',  ( 0.000000000000000000, -0.000000000000000000, 1.000000000000000000 ) ) ;
#20820=LINE ( 'NONE', #30005, #55843 ) ;
#20821=AXIS2_PLACEMENT_3D ( 'NONE', #1437, #41389, #60390 ) ;
#20822=ORIENTED_EDGE ( 'NONE', *, *, #67670, .F. ) ;
#20823=ORIENTED_EDGE ( 'NONE', *, *, #114450, .F. ) ;
#20824=ADVANCED_FACE ( 'NONE', ( #79885 ), #125851, .T. ) ;
#20825=CONICAL_SURFACE ( 'NONE', #85568, 0.1000000000000002554, 0.003490658503988666988 ) ;
#20826=ORIENTED_EDGE ( 'NONE', *, *, #114042, .F. ) ;
#20827=LINE ( 'NONE', #3122, #103941 ) ;
#20828=AXIS2_PLACEMENT_3D ( 'NONE', #98983, #76772, #107517 ) ;
#20829=DIRECTION ( 'NONE',  ( 0.000000000000000000, 0.000000000000000000, -1.000000000000000000 ) ) ;
#20830=DIRECTION ( 'NONE',  ( -0.000000000000000000, -1.000000000000000000, -0.000000000000000000 ) ) ;
#20831=ORIENTED_EDGE ( 'NONE', *, *, #31680, .T. ) ;
#20832=EDGE_LOOP ( 'NONE', ( #64360, #95852, #4525, #13737 ) ) ;
#20833=ORIENTED_EDGE ( 'NONE', *, *, #117567, .T. ) ;
#20834=DIRECTION ( 'NONE',  ( 0.000000000000000000, 1.000000000000000000, 0.000000000000000000 ) ) ;
#20835=ORIENTED_EDGE ( 'NONE', *, *, #51487, .T. ) ;
#20836=DIRECTION ( 'NONE',  ( -0.000000000000000000, -1.000000000000000000, -0.000000000000000000 ) ) ;
#20837=DIRECTION ( 'NONE',  ( -0.000000000000000000, -1.000000000000000000, -0.000000000000000000 ) ) ;
#20838=DIRECTION ( 'NONE',  ( 0.000000000000000000, 0.000000000000000000, 1.000000000000000000 ) ) ;
#20839=DIRECTION ( 'NONE',  ( 0.000000000000000000, 0.000000000000000000, 1.000000000000000000 ) ) ;
#20840=CARTESIAN_POINT ( 'NONE',  ( 1.249999999999952038, 2.500000000000000000, 5.702370205355745014 ) ) ;
#20841=CIRCLE ( 'NONE', #125388, 0.09999999999999999167 ) ;
#20842=CARTESIAN_POINT ( 'NONE',  ( -13.54999999999999005, 2.500000000000000000, 2.611473670974877148 ) ) ;
#20843=CARTESIAN_POINT ( 'NONE',  ( -1.850000000000033840, 12.50000000000000000, 2.511473670974873507 ) ) ;
#20844=VERTEX_POINT ( 'NONE', #50422 ) ;
#20845=ORIENTED_EDGE ( 'NONE', *, *, #112935, .F. ) ;
#20846=DIRECTION ( 'NONE',  ( 0.000000000000000000, 1.000000000000000000, 0.000000000000000000 ) ) ;
#20847=DIRECTION ( 'NONE',  ( 0.000000000000000000, 0.000000000000000000, -1.000000000000000000 ) ) ;
#20848=ORIENTED_EDGE ( 'NONE', *, *, #100827, .F. ) ;
#20849=EDGE_LOOP ( 'NONE', ( #121215, #123301, #12505, #36728, #102631, #23065, #104870, #2466, #116863, #78782, #21989, #11648, #39065 ) ) ;
#20850=DIRECTION ( 'NONE',  ( -0.000000000000000000, 1.000000000000000000, -0.000000000000000000 ) ) ;
#20851=DIRECTION ( 'NONE',  ( -0.000000000000000000, -1.000000000000000000, -0.000000000000000000 ) ) ;
#20852=DIRECTION ( 'NONE',  ( 0.000000000000000000, -0.9999939076577903929, 0.003490651415223739937 ) ) ;
#20853=DIRECTION ( 'NONE',  ( 0.000000000000000000, 0.000000000000000000, 1.000000000000000000 ) ) ;
#20854=ADVANCED_FACE ( 'NONE', ( #68122 ), #128013, .T. ) ;
#20855=CARTESIAN_POINT ( 'NONE',  ( -1.900000000000034106, 2.500000000000000000, 0.4464101615137735513 ) ) ;
#20856=DIRECTION ( 'NONE',  ( 0.000000000000000000, 0.000000000000000000, 1.000000000000000000 ) ) ;
#20857=DIRECTION ( 'NONE',  ( 0.000000000000000000, 0.000000000000000000, 1.000000000000000000 ) ) ;
#20858=VECTOR ( 'NONE', #30015, 1000.000000000000000 ) ;
#20859=FACE_OUTER_BOUND ( 'NONE', #2781, .T. ) ;
#20861=ORIENTED_EDGE ( 'NONE', *, *, #111016, .F. ) ;
#20862=EDGE_LOOP ( 'NONE', ( #5491, #70455, #15556, #115935 ) ) ;
#20863=AXIS2_PLACEMENT_3D ( 'NONE', #97823, #76903, #46807 ) ;
#20864=AXIS2_PLACEMENT_3D ( 'NONE', #105766, #106399, #27191 ) ;
#20865=EDGE_LOOP ( 'NONE', ( #51869, #53400 ) ) ;
#20866=AXIS2_PLACEMENT_3D ( 'NONE', #108195, #6123, #86626 ) ;
#20867=EDGE_CURVE ( 'NONE', #107780, #7939, #115464, .T. ) ;
#20868=EDGE_LOOP ( 'NONE', ( #31081, #95699 ) ) ;
#20869=ORIENTED_EDGE ( 'NONE', *, *, #88633, .F. ) ;
#20870=EDGE_CURVE ( 'NONE', #4913, #47413, #70710, .T. ) ;
#20871=CARTESIAN_POINT ( 'NONE',  ( 8.349999999999919709, 12.50000000000000000, -2.792790559304616504 ) ) ;
#20872=DIRECTION ( 'NONE',  ( 0.000000000000000000, 0.000000000000000000, 1.000000000000000000 ) ) ;
#20873=VECTOR ( 'NONE', #27282, 1000.000000000000000 ) ;
#20874=CONICAL_SURFACE ( 'NONE', #24982, 0.09999999999999982514, 0.003490658503988666988 ) ;
#20875=EDGE_LOOP ( 'NONE', ( #53444, #64861 ) ) ;
#20876=FACE_OUTER_BOUND ( 'NONE', #72331, .T. ) ;
#20878=EDGE_CURVE ( 'NONE', #25375, #107896, #51090, .T. ) ;
#20879=DIRECTION ( 'NONE',  ( 0.000000000000000000, 0.000000000000000000, 1.000000000000000000 ) ) ;
#20880=DIRECTION ( 'NONE',  ( 0.000000000000000000, 1.000000000000000000, 0.000000000000000000 ) ) ;
#20881=EDGE_LOOP ( 'NONE', ( #103033, #86786, #2097, #114002 ) ) ;
#20882=EDGE_CURVE ( 'NONE', #107817, #79702, #41272, .T. ) ;
#20883=CARTESIAN_POINT ( 'NONE',  ( -7.900000000000011013, 12.50000000000000000, 5.022947341949748790 ) ) ;
#20884=CARTESIAN_POINT ( 'NONE',  ( -15.39999999999997904, 12.50000000000000000, -0.7579135962115893799 ) ) ;
#20885=ORIENTED_EDGE ( 'NONE', *, *, #22412, .T. ) ;
#20886=EDGE_LOOP ( 'NONE', ( #4899, #82580, #60703, #21145 ) ) ;
#20888=VERTEX_POINT ( 'NONE', #123655 ) ;
#20889=DIRECTION ( 'NONE',  ( 0.000000000000000000, 0.000000000000000000, 1.000000000000000000 ) ) ;
#20890=FACE_OUTER_BOUND ( 'NONE', #18574, .T. ) ;
#20891=CARTESIAN_POINT ( 'NONE',  ( -0.8500000000000386136, 2.500000000000000000, 1.572243186433545548 ) ) ;
#20892=AXIS2_PLACEMENT_3D ( 'NONE', #14592, #2197, #72892 ) ;
#20893=VECTOR ( 'NONE', #5485, 1000.000000000000000 ) ;
#20894=DIRECTION ( 'NONE',  ( 0.000000000000000000, -0.9999939076577903929, 0.003490651415223739937 ) ) ;
#20895=VERTEX_POINT ( 'NONE', #1954 ) ;
#20896=CARTESIAN_POINT ( 'NONE',  ( -3.100000000000028511, 2.500000000000000000, -3.983716857408426293 ) ) ;
#20897=CARTESIAN_POINT ( 'NONE',  ( -12.89999999999999147, 2.500000000000000000, 3.737306695894644371 ) ) ;
#20898=LINE ( 'NONE', #42488, #31699 ) ;
#20899=DIRECTION ( 'NONE',  ( 0.000000000000000000, -0.000000000000000000, 1.000000000000000000 ) ) ;
#20900=CIRCLE ( 'NONE', #66860, 0.1000000000000002554 ) ;
#20901=ORIENTED_EDGE ( 'NONE', *, *, #104937, .F. ) ;
#20902=ORIENTED_EDGE ( 'NONE', *, *, #42664, .F. ) ;
#20904=CARTESIAN_POINT ( 'NONE',  ( -0.8500000000000382805, 12.50000000000000000, -2.857883832488653741 ) ) ;
#20905=CARTESIAN_POINT ( 'NONE',  ( -7.950000000000016165, 2.500000000000000000, -6.495190528383297135 ) ) ;
#20906=FACE_BOUND ( 'NONE', #4883, .T. ) ;
#20907=AXIS2_PLACEMENT_3D ( 'NONE', #22394, #93060, #74053 ) ;
#20908=DIRECTION ( 'NONE',  ( -0.000000000000000000, -1.000000000000000000, -0.000000000000000000 ) ) ;
#20909=DIRECTION ( 'NONE',  ( 0.000000000000000000, 1.000000000000000000, 0.000000000000000000 ) ) ;
#20910=EDGE_CURVE ( 'NONE', #28738, #64836, #107162, .T. ) ;
#20911=CARTESIAN_POINT ( 'NONE',  ( 3.949999999999941558, 2.500000000000000000, -1.918653347947326004 ) ) ;
#20912=AXIS2_PLACEMENT_3D ( 'NONE', #30887, #108765, #1395 ) ;
#20913=AXIS2_PLACEMENT_3D ( 'NONE', #35408, #94303, #93675 ) ;
#20914=EDGE_CURVE ( 'NONE', #94964, #4541, #44477, .T. ) ;
#20915=EDGE_CURVE ( 'NONE', #98238, #63941, #56981, .T. ) ;
#20916=DIRECTION ( 'NONE',  ( -0.000000000000000000, -1.000000000000000000, -0.000000000000000000 ) ) ;
#20917=AXIS2_PLACEMENT_3D ( 'NONE', #126414, #117862, #79257 ) ;
#20918=DIRECTION ( 'NONE',  ( 0.000000000000000000, -0.000000000000000000, 1.000000000000000000 ) ) ;
#20919=EDGE_CURVE ( 'NONE', #30265, #119631, #123889, .T. ) ;
#20920=CARTESIAN_POINT ( 'NONE',  ( -14.14999999999998792, 2.500000000000000000, -1.472243186433547901 ) ) ;
#20921=EDGE_LOOP ( 'NONE', ( #54843, #44426 ) ) ;
#20922=AXIS2_PLACEMENT_3D ( 'NONE', #125684, #76604, #36038 ) ;
#20923=ADVANCED_FACE ( 'NONE', ( #104042 ), #61213, .T. ) ;
#20924=LINE ( 'NONE', #92223, #38674 ) ;
#20925=DIRECTION ( 'NONE',  ( 0.000000000000000000, -0.000000000000000000, 1.000000000000000000 ) ) ;
#20927=AXIS2_PLACEMENT_3D ( 'NONE', #82448, #80508, #61516 ) ;
#20928=EDGE_LOOP ( 'NONE', ( #90225, #73477 ) ) ;
#20929=ORIENTED_EDGE ( 'NONE', *, *, #43334, .T. ) ;
#20930=DIRECTION ( 'NONE',  ( 0.000000000000000000, -0.000000000000000000, 1.000000000000000000 ) ) ;
#20931=DIRECTION ( 'NONE',  ( 0.000000000000000000, 1.000000000000000000, 0.000000000000000000 ) ) ;
#20932=FACE_BOUND ( 'NONE', #13961, .T. ) ;
#20933=CARTESIAN_POINT ( 'NONE',  ( -9.999999999999969802, 12.50000000000000000, 4.330127018922196314 ) ) ;
#20934=EDGE_CURVE ( 'NONE', #8949, #15822, #94215, .T. ) ;
#20935=ADVANCED_FACE ( 'NONE', ( #13708 ), #27748, .T. ) ;
#20936=DIRECTION ( 'NONE',  ( 0.000000000000000000, 0.000000000000000000, 1.000000000000000000 ) ) ;
#20937=ORIENTED_EDGE ( 'NONE', *, *, #37308, .T. ) ;
#20938=CARTESIAN_POINT ( 'NONE',  ( 9.149999999999920419, 2.500000000000000000, -5.702370205355749455 ) ) ;
#20940=ORIENTED_EDGE ( 'NONE', *, *, #34948, .T. ) ;
#20941=CARTESIAN_POINT ( 'NONE',  ( -4.350000000000023626, 2.500000000000000000, 6.741600689897071952 ) ) ;
#20942=DIRECTION ( 'NONE',  ( 0.000000000000000000, 0.000000000000000000, 1.000000000000000000 ) ) ;
#20943=AXIS2_PLACEMENT_3D ( 'NONE', #52077, #41627, #80248 ) ;
#20944=CARTESIAN_POINT ( 'NONE',  ( -2.499999999999996003, 2.500000000000000000, -0.1000000000000022815 ) ) ;
#20945=CIRCLE ( 'NONE', #62811, 0.06509327318403745899 ) ;
#20946=DIRECTION ( 'NONE',  ( -0.000000000000000000, 1.000000000000000000, -0.000000000000000000 ) ) ;
#20947=EDGE_CURVE ( 'NONE', #40320, #86459, #111354, .T. ) ;
#20948=EDGE_LOOP ( 'NONE', ( #22990, #24224, #98646, #53921 ) ) ;
#20949=CARTESIAN_POINT ( 'NONE',  ( 8.549999999999922551, 2.500000000000000000, -6.148780366869526226 ) ) ;
#20950=VECTOR ( 'NONE', #22517, 1000.000000000000000 ) ;
#20951=AXIS2_PLACEMENT_3D ( 'NONE', #103017, #102391, #103684 ) ;
#20952=LINE ( 'NONE', #62183, #62241 ) ;
#20953=FACE_OUTER_BOUND ( 'NONE', #11613, .T. ) ;
#20954=EDGE_LOOP ( 'NONE', ( #80150, #43283 ) ) ;
#20955=ORIENTED_EDGE ( 'NONE', *, *, #34648, .T. ) ;
#20957=EDGE_LOOP ( 'NONE', ( #46445, #100482 ) ) ;
#20958=LINE ( 'NONE', #42556, #28418 ) ;
#20959=CIRCLE ( 'NONE', #117087, 0.1000000000000002554 ) ;
#20960=CARTESIAN_POINT ( 'NONE',  ( -10.00000000000000711, 12.50000000000000000, -3.702399969078682851 ) ) ;
#20961=DIRECTION ( 'NONE',  ( 0.000000000000000000, 0.000000000000000000, 1.000000000000000000 ) ) ;
#20962=VERTEX_POINT ( 'NONE', #14350 ) ;
#20963=FACE_OUTER_BOUND ( 'NONE', #106378, .T. ) ;
#20964=DIRECTION ( 'NONE',  ( 0.000000000000000000, 0.000000000000000000, 1.000000000000000000 ) ) ;
#20965=DIRECTION ( 'NONE',  ( 0.000000000000000000, 1.000000000000000000, 0.000000000000000000 ) ) ;
#20966=PLANE ( 'NONE',  #87275 ) ;
#20967=CARTESIAN_POINT ( 'NONE',  ( -0.8000000000000376810, 12.50000000000000000, -4.330127018922201643 ) ) ;
#20968=FACE_OUTER_BOUND ( 'NONE', #9038, .T. ) ;
#20969=ORIENTED_EDGE ( 'NONE', *, *, #123836, .T. ) ;
#20970=EDGE_CURVE ( 'NONE', #72461, #92222, #13060, .T. ) ;
#20971=ORIENTED_EDGE ( 'NONE', *, *, #26086, .F. ) ;
#20972=DIRECTION ( 'NONE',  ( 0.000000000000000000, 0.000000000000000000, -1.000000000000000000 ) ) ;
#20973=ORIENTED_EDGE ( 'NONE', *, *, #53627, .T. ) ;
#20974=CARTESIAN_POINT ( 'NONE',  ( -0.6500000000000398792, 12.50000000000000000, -2.446380397790840266 ) ) ;
#20975=ORIENTED_EDGE ( 'NONE', *, *, #41783, .F. ) ;
#20976=ORIENTED_EDGE ( 'NONE', *, *, #58616, .F. ) ;
#20977=ORIENTED_EDGE ( 'NONE', *, *, #11829, .F. ) ;
#20978=CARTESIAN_POINT ( 'NONE',  ( 17.50000000000000000, -2.500000000000000000, -3.999999999999998224 ) ) ;
#20979=CONICAL_SURFACE ( 'NONE', #94136, 0.1000000000000000472, 0.003490658503988666988 ) ;
#20980=CARTESIAN_POINT ( 'NONE',  ( 2.699999999999947331, 12.50000000000000000, -0.3464101615137783474 ) ) ;
#20981=AXIS2_PLACEMENT_3D ( 'NONE', #69271, #29381, #31319 ) ;
#20982=DIRECTION ( 'NONE',  ( 0.000000000000000000, 1.000000000000000000, 0.000000000000000000 ) ) ;
#20984=DIRECTION ( 'NONE',  ( 0.000000000000000000, 0.000000000000000000, 1.000000000000000000 ) ) ;
#20985=CARTESIAN_POINT ( 'NONE',  ( -1.900000000000034106, 12.50000000000000000, 0.3464101615137735735 ) ) ;
#20987=DIRECTION ( 'NONE',  ( -0.000000000000000000, -1.000000000000000000, -0.000000000000000000 ) ) ;
#20988=CARTESIAN_POINT ( 'NONE',  ( -10.45000000000000107, 2.500000000000000000, 2.165063509461097713 ) ) ;
#20989=FACE_OUTER_BOUND ( 'NONE', #58232, .T. ) ;
#20990=VECTOR ( 'NONE', #20894, 1000.000000000000000 ) ;
#20991=EDGE_LOOP ( 'NONE', ( #114354, #124895, #103496, #2214 ) ) ;
#20992=CARTESIAN_POINT ( 'NONE',  ( -10.45000000000000107, 12.50000000000000000, 6.560283801567334372 ) ) ;
#20993=ORIENTED_EDGE ( 'NONE', *, *, #30138, .T. ) ;
#20994=ORIENTED_EDGE ( 'NONE', *, *, #126123, .T. ) ;
#20995=LINE ( 'NONE', #58368, #41975 ) ;
#20996=CARTESIAN_POINT ( 'NONE',  ( 6.899999999999928413, 2.500000000000000000, 4.776537180435972196 ) ) ;
#20997=CIRCLE ( 'NONE', #66948, 0.09999999999999982514 ) ;
#20998=DIRECTION ( 'NONE',  ( 0.000000000000000000, 0.000000000000000000, -1.000000000000000000 ) ) ;
#20999=VECTOR ( 'NONE', #52301, 1000.000000000000000 ) ;
#21000=DIRECTION ( 'NONE',  ( 0.000000000000000000, 0.000000000000000000, 1.000000000000000000 ) ) ;
#21001=DIRECTION ( 'NONE',  ( -0.000000000000000000, 1.000000000000000000, -0.000000000000000000 ) ) ;
#21002=DIRECTION ( 'NONE',  ( 0.000000000000000000, 0.000000000000000000, 1.000000000000000000 ) ) ;
#21003=ORIENTED_EDGE ( 'NONE', *, *, #103168, .F. ) ;
#21004=AXIS2_PLACEMENT_3D ( 'NONE', #91581, #112520, #21553 ) ;
#21005=VERTEX_POINT ( 'NONE', #73281 ) ;
#21006=DIRECTION ( 'NONE',  ( 0.000000000000000000, 0.000000000000000000, 1.000000000000000000 ) ) ;
#21007=ADVANCED_FACE ( 'NONE', ( #112581 ), #25589, .T. ) ;
#21009=LINE ( 'NONE', #53549, #46255 ) ;
#21010=AXIS2_PLACEMENT_3D ( 'NONE', #124765, #95946, #27849 ) ;
#21011=VERTEX_POINT ( 'NONE', #22910 ) ;
#21012=EDGE_CURVE ( 'NONE', #91607, #71034, #86227, .T. ) ;
#21013=ORIENTED_EDGE ( 'NONE', *, *, #76937, .T. ) ;
#21014=EDGE_CURVE ( 'NONE', #87232, #5884, #121097, .T. ) ;
#21015=CARTESIAN_POINT ( 'NONE',  ( -0.4000000000000396572, 2.500000000000000000, 4.230127018922196669 ) ) ;
#21016=DIRECTION ( 'NONE',  ( 0.000000000000000000, 0.000000000000000000, 1.000000000000000000 ) ) ;
#21017=DIRECTION ( 'NONE',  ( 0.000000000000000000, 0.000000000000000000, -1.000000000000000000 ) ) ;
#21018=DIRECTION ( 'NONE',  ( 0.000000000000000000, 1.000000000000000000, 0.000000000000000000 ) ) ;
#21019=EDGE_CURVE ( 'NONE', #122356, #108389, #8862, .T. ) ;
#21020=CARTESIAN_POINT ( 'NONE',  ( 87.50000000000001421, -3.974992050023846257, 6.359987280038160939 ) ) ;
#21021=ADVANCED_FACE ( 'NONE', ( #113199 ), #31981, .T. ) ;
#21022=VERTEX_POINT ( 'NONE', #53647 ) ;
#21023=CARTESIAN_POINT ( 'NONE',  ( -0.8500000000000390576, 2.500000000000000000, -2.065063509461102065 ) ) ;
#21024=CARTESIAN_POINT ( 'NONE',  ( 8.549999999999924327, 12.50000000000000000, 1.753560074763284016 ) ) ;
#21025=EDGE_CURVE ( 'NONE', #73329, #97417, #59063, .T. ) ;
#21026=DIRECTION ( 'NONE',  ( 0.000000000000000000, 0.000000000000000000, 1.000000000000000000 ) ) ;
#21027=ADVANCED_FACE ( 'NONE', ( #83754 ), #125943, .T. ) ;
#21029=CARTESIAN_POINT ( 'NONE',  ( -3.950000000000028155, 12.50000000000000000, -6.841600689897077814 ) ) ;
#21030=CARTESIAN_POINT ( 'NONE',  ( 5.849999999999931255, 12.50000000000000000, 2.922977105672686982 ) ) ;
#21031=ORIENTED_EDGE ( 'NONE', *, *, #29296, .T. ) ;
#21032=VERTEX_POINT ( 'NONE', #34677 ) ;
#21033=ORIENTED_EDGE ( 'NONE', *, *, #56808, .T. ) ;
#21034=CONICAL_SURFACE ( 'NONE', #119318, 0.1000000000000000472, 0.003490658503988666988 ) ;
#21035=CARTESIAN_POINT ( 'NONE',  ( -1.450000000000035039, 2.500000000000000000, -2.511473670974877948 ) ) ;
#21036=CIRCLE ( 'NONE', #60756, 0.09999999999999982514 ) ;
#21037=EDGE_CURVE ( 'NONE', #48425, #585, #4749, .T. ) ;
#21038=ORIENTED_EDGE ( 'NONE', *, *, #31419, .F. ) ;
#21039=CARTESIAN_POINT ( 'NONE',  ( 17.50000000000000000, -2.481874935395255832, 3.264429721014085573 ) ) ;
#21040=DIRECTION ( 'NONE',  ( 0.000000000000000000, 0.000000000000000000, -1.000000000000000000 ) ) ;
#21041=EDGE_LOOP ( 'NONE', ( #125393, #78779 ) ) ;
#21042=DIRECTION ( 'NONE',  ( 0.000000000000000000, 0.000000000000000000, 1.000000000000000000 ) ) ;
#21043=DIRECTION ( 'NONE',  ( 0.000000000000000000, 1.000000000000000000, 0.000000000000000000 ) ) ;
#21044=CARTESIAN_POINT ( 'NONE',  ( -9.350000000000006750, 12.50000000000000000, -2.576566944158915184 ) ) ;
#21045=DIRECTION ( 'NONE',  ( 0.000000000000000000, 1.000000000000000000, 0.000000000000000000 ) ) ;
#21046=DIRECTION ( 'NONE',  ( -0.000000000000000000, -1.000000000000000000, -0.000000000000000000 ) ) ;
#21047=ORIENTED_EDGE ( 'NONE', *, *, #38361, .T. ) ;
#21048=DIRECTION ( 'NONE',  ( -4.274815082592931898E-19, -0.9999939076577903929, -0.003490651415223739937 ) ) ;
#21049=CARTESIAN_POINT ( 'NONE',  ( 4.549999999999937650, 12.50000000000000000, 2.099970236277060032 ) ) ;
#21050=DIRECTION ( 'NONE',  ( 0.000000000000000000, 1.000000000000000000, 0.000000000000000000 ) ) ;
#21051=CARTESIAN_POINT ( 'NONE',  ( -9.400000000000007461, 2.500000000000000000, 4.083716857408420609 ) ) ;
#21052=VERTEX_POINT ( 'NONE', #116418 ) ;
#21053=VERTEX_POINT ( 'NONE', #35311 ) ;
#21054=EDGE_CURVE ( 'NONE', #118622, #71534, #26129, .T. ) ;
#21055=PLANE ( 'NONE',  #119115 ) ;
#21056=FACE_OUTER_BOUND ( 'NONE', #67370, .T. ) ;
#21057=DIRECTION ( 'NONE',  ( 0.000000000000000000, 0.000000000000000000, 1.000000000000000000 ) ) ;
#21058=EDGE_CURVE ( 'NONE', #2492, #58787, #109220, .T. ) ;
#21059=ORIENTED_EDGE ( 'NONE', *, *, #55612, .F. ) ;
#21060=VECTOR ( 'NONE', #85729, 1000.000000000000000 ) ;
#21061=CARTESIAN_POINT ( 'NONE',  ( -3.350000000000028955, 2.500000000000000000, 7.188010851410848723 ) ) ;
#21062=AXIS2_PLACEMENT_3D ( 'NONE', #118881, #31163, #59990 ) ;
#21063=ADVANCED_FACE ( 'NONE', ( #115115 ), #100897, .T. ) ;
#21064=CARTESIAN_POINT ( 'NONE',  ( -11.44999999999999751, 12.50000000000000000, 2.511473670974873507 ) ) ;
#21065=ORIENTED_EDGE ( 'NONE', *, *, #53088, .F. ) ;
#21066=LINE ( 'NONE', #100913, #126389 ) ;
#21067=ADVANCED_FACE ( 'NONE', ( #66675 ), #19332, .T. ) ;
#21068=ORIENTED_EDGE ( 'NONE', *, *, #96438, .F. ) ;
#21069=CIRCLE ( 'NONE', #6376, 0.1000000000000002554 ) ;
#21070=CARTESIAN_POINT ( 'NONE',  ( 11.69999999999990870, 12.50000000000000000, -4.330127018922201643 ) ) ;
#21072=AXIS2_PLACEMENT_3D ( 'NONE', #41310, #111293, #121137 ) ;
#21073=EDGE_CURVE ( 'NONE', #83615, #89926, #52792, .T. ) ;
#21074=ADVANCED_FACE ( 'NONE', ( #45774 ), #54925, .T. ) ;
#21075=ORIENTED_EDGE ( 'NONE', *, *, #45619, .F. ) ;
#21076=DIRECTION ( 'NONE',  ( 0.000000000000000000, 1.000000000000000000, 0.000000000000000000 ) ) ;
#21077=FACE_OUTER_BOUND ( 'NONE', #112767, .T. ) ;
#21078=ORIENTED_EDGE ( 'NONE', *, *, #100341, .T. ) ;
#21080=DIRECTION ( 'NONE',  ( 0.000000000000000000, 0.000000000000000000, -1.000000000000000000 ) ) ;
#21081=DIRECTION ( 'NONE',  ( 0.000000000000000000, 1.000000000000000000, 0.000000000000000000 ) ) ;
#21082=ORIENTED_EDGE ( 'NONE', *, *, #40699, .F. ) ;
#21083=ADVANCED_FACE ( 'NONE', ( #107254 ), #57524, .T. ) ;
#21084=CIRCLE ( 'NONE', #110956, 0.06509327318403745899 ) ;
#21085=CARTESIAN_POINT ( 'NONE',  ( -4.251297162942325111E-14, 2.500000000000000000, -3.737306695894649700 ) ) ;
#21088=CARTESIAN_POINT ( 'NONE',  ( 11.89999999999990798, 2.500000000000000000, -3.883716857408426648 ) ) ;
#21089=CARTESIAN_POINT ( 'NONE',  ( 9.799999999999917222, 2.500000000000000000, 0.2464101615137735679 ) ) ;
#21090=DIRECTION ( 'NONE',  ( 0.000000000000000000, 0.000000000000000000, 1.000000000000000000 ) ) ;
#21091=PLANE ( 'NONE',  #24325 ) ;
#21092=DIRECTION ( 'NONE',  ( 0.000000000000000000, 1.000000000000000000, 0.000000000000000000 ) ) ;
#21093=CIRCLE ( 'NONE', #46140, 0.06509327318403745899 ) ;
#21094=EDGE_LOOP ( 'NONE', ( #110494, #12121, #112401, #25392 ) ) ;
#21095=ORIENTED_EDGE ( 'NONE', *, *, #116890, .F. ) ;
#21096=CARTESIAN_POINT ( 'NONE',  ( 3.949999999999941558, 12.50000000000000000, -1.818653347947326138 ) ) ;
#21097=EDGE_LOOP ( 'NONE', ( #95419, #33687, #122643, #2681 ) ) ;
#21098=AXIS2_PLACEMENT_3D ( 'NONE', #61185, #81473, #33658 ) ;
#21099=CARTESIAN_POINT ( 'NONE',  ( 0.6499999999999543920, 2.500000000000000000, 6.841600689897072485 ) ) ;
#21100=FACE_OUTER_BOUND ( 'NONE', #76360, .T. ) ;
#21101=DIRECTION ( 'NONE',  ( 0.000000000000000000, 0.000000000000000000, -1.000000000000000000 ) ) ;
#21102=ORIENTED_EDGE ( 'NONE', *, *, #71190, .F. ) ;
#21103=ORIENTED_EDGE ( 'NONE', *, *, #83127, .F. ) ;
#21104=FACE_BOUND ( 'NONE', #82961, .T. ) ;
#21106=ADVANCED_FACE ( 'NONE', ( #46391 ), #71673, .T. ) ;
#21107=DIRECTION ( 'NONE',  ( 0.000000000000000000, 0.000000000000000000, 1.000000000000000000 ) ) ;
#21109=CARTESIAN_POINT ( 'NONE',  ( 1.899999999999951283, 2.500000000000000000, -3.883716857408426648 ) ) ;
#21110=CARTESIAN_POINT ( 'NONE',  ( -1.850000000000033396, 12.50000000000000000, -1.818653347947325916 ) ) ;
#21111=FACE_OUTER_BOUND ( 'NONE', #105457, .T. ) ;
#21112=CARTESIAN_POINT ( 'NONE',  ( 14.99999999999992895, 2.500000000000000000, 0.09999999999999772959 ) ) ;
#21113=DIRECTION ( 'NONE',  ( -0.000000000000000000, 1.000000000000000000, -0.000000000000000000 ) ) ;
#21114=LINE ( 'NONE', #834, #83338 ) ;
#21115=DIRECTION ( 'NONE',  ( 0.000000000000000000, 1.000000000000000000, 0.000000000000000000 ) ) ;
#21116=CARTESIAN_POINT ( 'NONE',  ( -4.150000000000028777, 2.500000000000000000, -5.702370205355749455 ) ) ;
#21117=DIRECTION ( 'NONE',  ( 0.000000000000000000, -0.9999939076577903929, 0.003490651415223739937 ) ) ;
#21118=ORIENTED_EDGE ( 'NONE', *, *, #26445, .F. ) ;
#21119=EDGE_LOOP ( 'NONE', ( #94408, #27801, #79848, #41177 ) ) ;
#21120=ADVANCED_FACE ( 'NONE', ( #105969 ), #15307, .T. ) ;
#21122=ORIENTED_EDGE ( 'NONE', *, *, #110702, .T. ) ;
#21123=DIRECTION ( 'NONE',  ( -0.000000000000000000, -1.000000000000000000, -0.000000000000000000 ) ) ;
#21124=AXIS2_PLACEMENT_3D ( 'NONE', #29241, #77666, #37756 ) ;
#21125=CARTESIAN_POINT ( 'NONE',  ( 6.249999999999932498, 2.500000000000000000, 5.802370205355744659 ) ) ;
#21126=VECTOR ( 'NONE', #91204, 1000.000000000000000 ) ;
#21127=VECTOR ( 'NONE', #68321, 1000.000000000000000 ) ;
#21128=ORIENTED_EDGE ( 'NONE', *, *, #13931, .T. ) ;
#21129=ORIENTED_EDGE ( 'NONE', *, *, #39254, .T. ) ;
#21130=ORIENTED_EDGE ( 'NONE', *, *, #79562, .F. ) ;
#21132=CIRCLE ( 'NONE', #37852, 0.1000000000000002554 ) ;
#21133=DIRECTION ( 'NONE',  ( 0.000000000000000000, 1.000000000000000000, 0.000000000000000000 ) ) ;
#21134=FILL_AREA_STYLE_COLOUR ( '', #104099 ) ;
#21135=DIRECTION ( 'NONE',  ( 0.000000000000000000, 0.000000000000000000, 1.000000000000000000 ) ) ;
#21136=LINE ( 'NONE', #11960, #105691 ) ;
#21138=AXIS2_PLACEMENT_3D ( 'NONE', #10200, #40317, #80235 ) ;
#21139=CARTESIAN_POINT ( 'NONE',  ( 6.899999999999928413, 12.50000000000000000, -4.676537180435977881 ) ) ;
#21140=EDGE_CURVE ( 'NONE', #86566, #7480, #5175, .T. ) ;
#21141=EDGE_LOOP ( 'NONE', ( #107816, #10787, #91477, #13781 ) ) ;
#21142=LINE ( 'NONE', #123224, #91447 ) ;
#21143=VERTEX_POINT ( 'NONE', #25454 ) ;
#21144=ORIENTED_EDGE ( 'NONE', *, *, #101586, .T. ) ;
#21145=ORIENTED_EDGE ( 'NONE', *, *, #117072, .F. ) ;
#21146=CARTESIAN_POINT ( 'NONE',  ( 10.79999999999991012, 2.500000000000000000, 4.230127018922196669 ) ) ;
#21147=VERTEX_POINT ( 'NONE', #117053 ) ;
#21148=ORIENTED_EDGE ( 'NONE', *, *, #5521, .T. ) ;
#21149=ORIENTED_EDGE ( 'NONE', *, *, #112109, .T. ) ;
#21150=DIRECTION ( 'NONE',  ( 0.000000000000000000, 0.000000000000000000, 1.000000000000000000 ) ) ;
#21152=DIRECTION ( 'NONE',  ( 0.000000000000000000, 0.000000000000000000, -1.000000000000000000 ) ) ;
#21153=PLANE ( 'NONE',  #14384 ) ;
#21154=CARTESIAN_POINT ( 'NONE',  ( 15.19999999999989093, 2.500000000000000000, 0.3464101615137735735 ) ) ;
#21155=CARTESIAN_POINT ( 'NONE',  ( 9.349999999999919709, 12.50000000000000000, 2.446380397790835826 ) ) ;
#21156=DIRECTION ( 'NONE',  ( 0.000000000000000000, 0.000000000000000000, 1.000000000000000000 ) ) ;
#21157=FACE_OUTER_BOUND ( 'NONE', #60080, .T. ) ;
#21158=AXIS2_PLACEMENT_3D ( 'NONE', #25513, #83801, #85089 ) ;
#21159=CONICAL_SURFACE ( 'NONE', #77505, 0.1000000000000002554, 0.003490658503988666988 ) ;
#21160=ORIENTED_EDGE ( 'NONE', *, *, #126738, .T. ) ;
#21161=DIRECTION ( 'NONE',  ( -0.000000000000000000, 1.000000000000000000, -0.000000000000000000 ) ) ;
#21162=EDGE_CURVE ( 'NONE', #79172, #108104, #645, .T. ) ;
#21163=VERTEX_POINT ( 'NONE', #105330 ) ;
#21164=DIRECTION ( 'NONE',  ( -0.000000000000000000, 1.000000000000000000, -0.000000000000000000 ) ) ;
#21165=PLANE ( 'NONE',  #37767 ) ;
#21166=ORIENTED_EDGE ( 'NONE', *, *, #116959, .F. ) ;
#21167=LINE ( 'NONE', #10682, #2870 ) ;
#21168=DIRECTION ( 'NONE',  ( -0.000000000000000000, 1.000000000000000000, -0.000000000000000000 ) ) ;
#21169=ORIENTED_EDGE ( 'NONE', *, *, #111178, .T. ) ;
#21170=VECTOR ( 'NONE', #75938, 1000.000000000000000 ) ;
#21171=EDGE_CURVE ( 'NONE', #1500, #112120, #27386, .T. ) ;
#21172=AXIS2_PLACEMENT_3D ( 'NONE', #121770, #32137, #53688 ) ;
#21173=CARTESIAN_POINT ( 'NONE',  ( 0.4499999999999552136, 12.50000000000000000, 6.495190528383297135 ) ) ;
#21174=ORIENTED_EDGE ( 'NONE', *, *, #16821, .T. ) ;
#21175=ADVANCED_FACE ( 'NONE', ( #6440 ), #63364, .T. ) ;
#21176=EDGE_CURVE ( 'NONE', #44930, #81872, #73815, .T. ) ;
#21177=VERTEX_POINT ( 'NONE', #78468 ) ;
#21178=DIRECTION ( 'NONE',  ( -4.274815082592931898E-19, -0.9999939076577903929, -0.003490651415223739937 ) ) ;
#21179=DIRECTION ( 'NONE',  ( -0.000000000000000000, 1.000000000000000000, -0.000000000000000000 ) ) ;
#21180=EDGE_CURVE ( 'NONE', #15629, #109700, #20817, .T. ) ;
#21181=LINE ( 'NONE', #61109, #23019 ) ;
#21182=EDGE_CURVE ( 'NONE', #7665, #12607, #88232, .T. ) ;
#21183=CARTESIAN_POINT ( 'NONE',  ( 7.499999999999927169, 12.50000000000000000, 3.702399969078682407 ) ) ;
#21184=AXIS2_PLACEMENT_3D ( 'NONE', #100443, #99805, #12055 ) ;
#21185=CARTESIAN_POINT ( 'NONE',  ( -13.74999999999998757, 12.50000000000000000, -2.857883832488651521 ) ) ;
#21186=ORIENTED_EDGE ( 'NONE', *, *, #92232, .T. ) ;
#21187=CARTESIAN_POINT ( 'NONE',  ( 11.84999999999990372, 2.500000000000000000, 1.818653347947321475 ) ) ;
#21188=ADVANCED_FACE ( 'NONE', ( #98078 ), #27841, .T. ) ;
#21189=AXIS2_PLACEMENT_3D ( 'NONE', #13492, #53448, #81599 ) ;
#21190=ORIENTED_EDGE ( 'NONE', *, *, #113301, .T. ) ;
#21191=EDGE_CURVE ( 'NONE', #6403, #74808, #65399, .T. ) ;
#21192=PLANE ( 'NONE',  #121789 ) ;
#21193=LINE ( 'NONE', #60500, #104438 ) ;
#21194=EDGE_CURVE ( 'NONE', #93259, #26633, #39192, .T. ) ;
#21195=CONICAL_SURFACE ( 'NONE', #50524, 0.1000000000000002554, 0.003490658503988666988 ) ;
#21196=CIRCLE ( 'NONE', #50443, 0.1000000000000002554 ) ;
#21198=CARTESIAN_POINT ( 'NONE',  ( 0.1999999999999567124, 2.500000000000000000, -3.983716857408426293 ) ) ;
#21199=DIRECTION ( 'NONE',  ( -0.000000000000000000, -1.000000000000000000, -0.000000000000000000 ) ) ;
#21200=DIRECTION ( 'NONE',  ( 0.000000000000000000, 1.000000000000000000, 0.000000000000000000 ) ) ;
#21201=FACE_OUTER_BOUND ( 'NONE', #18361, .T. ) ;
#21202=DIRECTION ( 'NONE',  ( 0.000000000000000000, 0.000000000000000000, 1.000000000000000000 ) ) ;
#21203=VERTEX_POINT ( 'NONE', #119012 ) ;
#21204=DIRECTION ( 'NONE',  ( 0.000000000000000000, 0.000000000000000000, 1.000000000000000000 ) ) ;
#21205=CARTESIAN_POINT ( 'NONE',  ( 8.149999999999923972, 2.500000000000000000, 1.818653347947321475 ) ) ;
#21206=CARTESIAN_POINT ( 'NONE',  ( 2.499999999999983569, 2.500000000000000000, 0.09999999999999772959 ) ) ;
#21207=VERTEX_POINT ( 'NONE', #120308 ) ;
#21208=DIRECTION ( 'NONE',  ( 0.000000000000000000, 0.000000000000000000, -1.000000000000000000 ) ) ;
#21209=ORIENTED_EDGE ( 'NONE', *, *, #40731, .T. ) ;
#21210=ORIENTED_EDGE ( 'NONE', *, *, #55909, .T. ) ;
#21211=DIRECTION ( 'NONE',  ( 0.000000000000000000, 0.000000000000000000, 1.000000000000000000 ) ) ;
#21212=CONICAL_SURFACE ( 'NONE', #115182, 0.1000000000000002554, 0.003490658503988666988 ) ;
#21213=CIRCLE ( 'NONE', #71290, 0.1000000000000002554 ) ;
#21214=CIRCLE ( 'NONE', #44291, 0.06509327318403745899 ) ;
#21215=ORIENTED_EDGE ( 'NONE', *, *, #84329, .F. ) ;
#21216=LINE ( 'NONE', #42831, #60228 ) ;
#21217=DIRECTION ( 'NONE',  ( 0.000000000000000000, 0.000000000000000000, -1.000000000000000000 ) ) ;
#21218=CARTESIAN_POINT ( 'NONE',  ( 3.549999999999943867, 2.500000000000000000, -6.048780366869526581 ) ) ;
#21219=ORIENTED_EDGE ( 'NONE', *, *, #31131, .F. ) ;
#21220=VECTOR ( 'NONE', #73860, 1000.000000000000000 ) ;
#21221=CARTESIAN_POINT ( 'NONE',  ( -11.05000000000000071, 12.50000000000000000, 2.511473670974873507 ) ) ;
#21222=AXIS2_PLACEMENT_3D ( 'NONE', #20809, #60737, #120933 ) ;
#21223=CARTESIAN_POINT ( 'NONE',  ( -5.600000000000020073, 12.50000000000000000, 4.676537180435972552 ) ) ;
#21224=CARTESIAN_POINT ( 'NONE',  ( 11.84999999999990727, 2.500000000000000000, -1.718653347947326049 ) ) ;
#21225=EDGE_CURVE ( 'NONE', #124539, #105724, #29360, .T. ) ;
#21226=ORIENTED_EDGE ( 'NONE', *, *, #51644, .T. ) ;
#21227=EDGE_CURVE ( 'NONE', #83483, #111264, #94745, .T. ) ;
#21228=ORIENTED_EDGE ( 'NONE', *, *, #100647, .T. ) ;
#21229=EDGE_CURVE ( 'NONE', #73117, #123848, #38549, .T. ) ;
#21230=ORIENTED_EDGE ( 'NONE', *, *, #25929, .F. ) ;
#21231=FACE_OUTER_BOUND ( 'NONE', #81791, .T. ) ;
#21232=DIRECTION ( 'NONE',  ( 0.000000000000000000, 0.000000000000000000, -1.000000000000000000 ) ) ;
#21233=DIRECTION ( 'NONE',  ( -4.274815082592931898E-19, -0.9999939076577903929, -0.003490651415223739937 ) ) ;
#21234=FACE_BOUND ( 'NONE', #16402, .T. ) ;
#21235=EDGE_LOOP ( 'NONE', ( #57356, #45730, #57579, #42063 ) ) ;
#21236=DIRECTION ( 'NONE',  ( -0.000000000000000000, 1.000000000000000000, -0.000000000000000000 ) ) ;
#21237=FACE_OUTER_BOUND ( 'NONE', #5532, .T. ) ;
#21238=ORIENTED_EDGE ( 'NONE', *, *, #124652, .F. ) ;
#21239=ADVANCED_FACE ( 'NONE', ( #98710 ), #48789, .T. ) ;
#21240=DIRECTION ( 'NONE',  ( 0.000000000000000000, 0.000000000000000000, -1.000000000000000000 ) ) ;
#21241=CARTESIAN_POINT ( 'NONE',  ( 4.399999999999940847, 2.500000000000000000, -4.083716857408426826 ) ) ;
#21242=CARTESIAN_POINT ( 'NONE',  ( 7.099999999999925926, 2.500000000000000000, 0.5928203230275495006 ) ) ;
#21243=FACE_OUTER_BOUND ( 'NONE', #50703, .T. ) ;
#21245=DIRECTION ( 'NONE',  ( 0.000000000000000000, 0.000000000000000000, -1.000000000000000000 ) ) ;
#21246=DIRECTION ( 'NONE',  ( -0.000000000000000000, 1.000000000000000000, -0.000000000000000000 ) ) ;
#21247=CIRCLE ( 'NONE', #42191, 0.06509327318403745899 ) ;
#21248=CIRCLE ( 'NONE', #6543, 0.06509327318403743123 ) ;
#21249=EDGE_LOOP ( 'NONE', ( #25721, #96469, #19698, #27920 ) ) ;
#21250=VERTEX_POINT ( 'NONE', #109174 ) ;
#21251=ORIENTED_EDGE ( 'NONE', *, *, #60918, .T. ) ;
#21252=ORIENTED_EDGE ( 'NONE', *, *, #26654, .F. ) ;
#21253=DIRECTION ( 'NONE',  ( 0.000000000000000000, -0.9999939076577903929, 0.003490651415223739937 ) ) ;
#21254=CARTESIAN_POINT ( 'NONE',  ( 11.44999999999990692, 2.500000000000000000, -6.941600689897078347 ) ) ;
#21255=EDGE_LOOP ( 'NONE', ( #114836, #129556 ) ) ;
#21256=FACE_BOUND ( 'NONE', #58576, .T. ) ;
#21258=CONICAL_SURFACE ( 'NONE', #29580, 0.09999999999999999167, 0.003490658503988666988 ) ;
#21259=CARTESIAN_POINT ( 'NONE',  ( 1.699999999999951994, 12.50000000000000000, -2.276824562219559311E-15 ) ) ;
#21260=CONICAL_SURFACE ( 'NONE', #46296, 0.1000000000000000056, 0.003490658503988666988 ) ;
#21261=DIRECTION ( 'NONE',  ( 0.000000000000000000, -0.9999939076577903929, 0.003490651415223739937 ) ) ;
#21262=CIRCLE ( 'NONE', #77687, 0.06509327318403745899 ) ;
#21263=DIRECTION ( 'NONE',  ( -4.274815082592931898E-19, -0.9999939076577903929, -0.003490651415223739937 ) ) ;
#21264=DIRECTION ( 'NONE',  ( 0.000000000000000000, 0.000000000000000000, 1.000000000000000000 ) ) ;
#21265=DIRECTION ( 'NONE',  ( -0.000000000000000000, -1.000000000000000000, -0.000000000000000000 ) ) ;
#21266=CARTESIAN_POINT ( 'NONE',  ( 6.049999999999934097, 2.500000000000000000, -6.048780366869526581 ) ) ;
#21267=DIRECTION ( 'NONE',  ( 0.000000000000000000, 1.000000000000000000, 0.000000000000000000 ) ) ;
#21268=CARTESIAN_POINT ( 'NONE',  ( -3.100000000000028955, 12.50000000000000000, 3.983716857408420964 ) ) ;
#21269=ORIENTED_EDGE ( 'NONE', *, *, #16029, .T. ) ;
#21270=CIRCLE ( 'NONE', #60980, 0.1000000000000002554 ) ;
#21271=EDGE_LOOP ( 'NONE', ( #86031, #70242 ) ) ;
#21273=CONICAL_SURFACE ( 'NONE', #35948, 0.1000000000000000472, 0.003490658503988666988 ) ;
#21275=EDGE_LOOP ( 'NONE', ( #71038, #99531 ) ) ;
#21276=EDGE_CURVE ( 'NONE', #101165, #72896, #57088, .T. ) ;
#21277=ORIENTED_EDGE ( 'NONE', *, *, #114808, .T. ) ;
#21278=EDGE_LOOP ( 'NONE', ( #95580, #91044, #118137, #24867 ) ) ;
#21279=AXIS2_PLACEMENT_3D ( 'NONE', #88140, #90086, #47613 ) ;
#21280=CONICAL_SURFACE ( 'NONE', #75643, 0.1000000000000002554, 0.003490658503988666988 ) ;
#21281=CARTESIAN_POINT ( 'NONE',  ( -3.950000000000028155, 2.500000000000000000, -6.841600689897077814 ) ) ;
#21282=VERTEX_POINT ( 'NONE', #9045 ) ;
#21283=CONICAL_SURFACE ( 'NONE', #38007, 0.09999999999999982514, 0.003490658503988666988 ) ;
#21284=CARTESIAN_POINT ( 'NONE',  ( 17.37282530749033427, 0.4689596142739222984, 5.357821376857530460 ) ) ;
#21285=AXIS2_PLACEMENT_3D ( 'NONE', #115919, #36734, #24962 ) ;
#21286=CARTESIAN_POINT ( 'NONE',  ( 16.56576425164984201, -2.499999999999999556, 6.084390597446047266 ) ) ;
#21287=FACE_OUTER_BOUND ( 'NONE', #115482, .T. ) ;
#21288=DIRECTION ( 'NONE',  ( 0.000000000000000000, 0.000000000000000000, 1.000000000000000000 ) ) ;
#21289=ADVANCED_FACE ( 'NONE', ( #58180 ), #52901, .T. ) ;
#21292=ORIENTED_EDGE ( 'NONE', *, *, #14346, .T. ) ;
#21293=ORIENTED_EDGE ( 'NONE', *, *, #46314, .F. ) ;
#21294=LINE ( 'NONE', #71692, #119981 ) ;
#21295=FACE_OUTER_BOUND ( 'NONE', #101056, .T. ) ;
#21296=DIRECTION ( 'NONE',  ( -0.000000000000000000, -1.000000000000000000, -0.000000000000000000 ) ) ;
#21297=ADVANCED_FACE ( 'NONE', ( #48339 ), #2697, .T. ) ;
#21298=ORIENTED_EDGE ( 'NONE', *, *, #113743, .T. ) ;
#21299=ORIENTED_EDGE ( 'NONE', *, *, #25060, .F. ) ;
#21300=DIRECTION ( 'NONE',  ( 0.000000000000000000, 1.000000000000000000, 0.000000000000000000 ) ) ;
#21301=CARTESIAN_POINT ( 'NONE',  ( 4.149999999999938183, 12.50000000000000000, 2.165063509461097713 ) ) ;
#21302=DIRECTION ( 'NONE',  ( -0.000000000000000000, -1.000000000000000000, -0.000000000000000000 ) ) ;
#21303=AXIS2_PLACEMENT_3D ( 'NONE', #110581, #20916, #51039 ) ;
#21304=FACE_OUTER_BOUND ( 'NONE', #46068, .T. ) ;
#21305=VERTEX_POINT ( 'NONE', #89550 ) ;
#21306=AXIS2_PLACEMENT_3D ( 'NONE', #120012, #40829, #31012 ) ;
#21307=CARTESIAN_POINT ( 'NONE',  ( -13.14999999999999147, 2.500000000000000000, -2.611473670974875372 ) ) ;
#21308=VERTEX_POINT ( 'NONE', #99384 ) ;
#21309=CARTESIAN_POINT ( 'NONE',  ( 8.299999999999922551, 2.500000000000000000, -4.430127018922202176 ) ) ;
#21310=VERTEX_POINT ( 'NONE', #9706 ) ;
#21311=DIRECTION ( 'NONE',  ( 0.000000000000000000, 0.000000000000000000, -1.000000000000000000 ) ) ;
#21312=AXIS2_PLACEMENT_3D ( 'NONE', #107430, #112904, #86494 ) ;
#21313=EDGE_CURVE ( 'NONE', #62304, #127558, #8960, .T. ) ;
#21314=CARTESIAN_POINT ( 'NONE',  ( 21.23528140090950345, -2.699413673072312392, 2.293764360948889802 ) ) ;
#21315=CARTESIAN_POINT ( 'NONE',  ( -10.65000000000000391, 2.500000000000000000, -1.918653347947322230 ) ) ;
#21316=AXIS2_PLACEMENT_3D ( 'NONE', #107732, #72970, #71674 ) ;
#21317=CIRCLE ( 'NONE', #79812, 0.06509327318403745899 ) ;
#21318=DIRECTION ( 'NONE',  ( 0.000000000000000000, 0.000000000000000000, 1.000000000000000000 ) ) ;
#21319=ORIENTED_EDGE ( 'NONE', *, *, #58873, .T. ) ;
#21320=VECTOR ( 'NONE', #14155, 1000.000000000000000 ) ;
#21321=ADVANCED_FACE ( 'NONE', ( #20168 ), #60116, .T. ) ;
#21322=DIRECTION ( 'NONE',  ( 0.000000000000000000, -0.9999939076577903929, 0.003490651415223739937 ) ) ;
#21323=FACE_OUTER_BOUND ( 'NONE', #80641, .T. ) ;
#21324=VERTEX_POINT ( 'NONE', #80390 ) ;
#21325=VERTEX_POINT ( 'NONE', #30649 ) ;
#21326=EDGE_CURVE ( 'NONE', #123620, #65442, #4849, .T. ) ;
#21327=EDGE_CURVE ( 'NONE', #32461, #45043, #90540, .T. ) ;
#21328=EDGE_LOOP ( 'NONE', ( #84882, #5881, #83242, #7708 ) ) ;
#21329=DIRECTION ( 'NONE',  ( -4.274815082592931898E-19, -0.9999939076577903929, -0.003490651415223739937 ) ) ;
#21330=DIRECTION ( 'NONE',  ( 0.000000000000000000, 0.000000000000000000, -1.000000000000000000 ) ) ;
#21331=DIRECTION ( 'NONE',  ( 0.000000000000000000, 1.000000000000000000, 0.000000000000000000 ) ) ;
#21332=EDGE_CURVE ( 'NONE', #70125, #92609, #92605, .T. ) ;
#21333=CARTESIAN_POINT ( 'NONE',  ( -9.550000000000006040, 12.50000000000000000, 2.099970236277060032 ) ) ;
#21335=DIRECTION ( 'NONE',  ( 0.000000000000000000, 1.000000000000000000, 0.000000000000000000 ) ) ;
#21336=CARTESIAN_POINT ( 'NONE',  ( -1.850000000000033396, 2.500000000000000000, -2.411473670974877859 ) ) ;
#21337=DIRECTION ( 'NONE',  ( -0.000000000000000000, 1.000000000000000000, -0.000000000000000000 ) ) ;
#21338=CARTESIAN_POINT ( 'NONE',  ( 11.64999999999990798, 2.500000000000000000, -2.957883832488653830 ) ) ;
#21339=LINE ( 'NONE', #34414, #77726 ) ;
#21340=ADVANCED_FACE ( 'NONE', ( #62685 ), #117707, .T. ) ;
#21341=EDGE_CURVE ( 'NONE', #44142, #107907, #59169, .T. ) ;
#21342=EDGE_CURVE ( 'NONE', #118459, #116018, #128209, .T. ) ;
#21343=AXIS2_PLACEMENT_3D ( 'NONE', #75413, #6022, #6639 ) ;
#21344=EDGE_CURVE ( 'NONE', #114635, #80732, #78023, .T. ) ;
#21345=ADVANCED_FACE ( 'NONE', ( #33849 ), #42445, .T. ) ;
#21346=EDGE_LOOP ( 'NONE', ( #125766, #25994 ) ) ;
#21347=DIRECTION ( 'NONE',  ( 0.000000000000000000, 1.000000000000000000, 0.000000000000000000 ) ) ;
#21348=ADVANCED_FACE ( 'NONE', ( #42396 ), #93422, .T. ) ;
#21350=DIRECTION ( 'NONE',  ( -4.274815082592931898E-19, -0.9999939076577903929, -0.003490651415223739937 ) ) ;
#21351=DIRECTION ( 'NONE',  ( 0.000000000000000000, 0.000000000000000000, -1.000000000000000000 ) ) ;
#21352=CIRCLE ( 'NONE', #71527, 0.1000000000000002554 ) ;
#21353=EDGE_CURVE ( 'NONE', #115594, #10073, #13153, .T. ) ;
#21354=AXIS2_PLACEMENT_3D ( 'NONE', #123372, #53998, #113556 ) ;
#21355=ORIENTED_EDGE ( 'NONE', *, *, #81486, .F. ) ;
#21356=LINE ( 'NONE', #31200, #109426 ) ;
#21357=VECTOR ( 'NONE', #55794, 1000.000000000000000 ) ;
#21358=CONICAL_SURFACE ( 'NONE', #23406, 0.1000000000000002554, 0.003490658503988666988 ) ;
#21359=CARTESIAN_POINT ( 'NONE',  ( 1.249999999999953815, 12.50000000000000000, 1.472243186433545459 ) ) ;
#21360=LINE ( 'NONE', #41675, #25374 ) ;
#21361=ORIENTED_EDGE ( 'NONE', *, *, #66682, .F. ) ;
#21362=CONICAL_SURFACE ( 'NONE', #52751, 0.1000000000000000472, 0.003490658503988666988 ) ;
#21363=ORIENTED_EDGE ( 'NONE', *, *, #60829, .F. ) ;
#21364=DIRECTION ( 'NONE',  ( 0.000000000000000000, 1.000000000000000000, 0.000000000000000000 ) ) ;
#21365=CIRCLE ( 'NONE', #42306, 0.06509327318403745899 ) ;
#21366=EDGE_LOOP ( 'NONE', ( #21082, #31921, #123930, #10180 ) ) ;
#21367=VECTOR ( 'NONE', #46051, 1000.000000000000000 ) ;
#21368=AXIS2_PLACEMENT_3D ( 'NONE', #106787, #127099, #17093 ) ;
#21369=ORIENTED_EDGE ( 'NONE', *, *, #31185, .F. ) ;
#21370=AXIS2_PLACEMENT_3D ( 'NONE', #108702, #50424, #8547 ) ;
#21371=DIRECTION ( 'NONE',  ( 0.000000000000000000, -0.9999939076577903929, 0.003490651415223739937 ) ) ;
#21372=CARTESIAN_POINT ( 'NONE',  ( -9.600000000000006750, 12.50000000000000000, -0.6928203230275542523 ) ) ;
#21373=DIRECTION ( 'NONE',  ( 0.000000000000000000, 1.000000000000000000, 0.000000000000000000 ) ) ;
#21374=CARTESIAN_POINT ( 'NONE',  ( 17.49862860983167323, 2.500000000000000000, -4.081131818001370704 ) ) ;
#21375=ORIENTED_EDGE ( 'NONE', *, *, #26333, .F. ) ;
#21376=CIRCLE ( 'NONE', #71555, 0.09999999999999982514 ) ;
#21377=CARTESIAN_POINT ( 'NONE',  ( -9.999999999999969802, 2.500000000000000000, 4.330127018922196314 ) ) ;
#21378=ORIENTED_EDGE ( 'NONE', *, *, #128425, .F. ) ;
#21379=DIRECTION ( 'NONE',  ( 0.000000000000000000, 0.000000000000000000, -1.000000000000000000 ) ) ;
#21380=DIRECTION ( 'NONE',  ( 0.000000000000000000, 0.000000000000000000, 1.000000000000000000 ) ) ;
#21381=ORIENTED_EDGE ( 'NONE', *, *, #50221, .F. ) ;
#21382=EDGE_CURVE ( 'NONE', #53076, #53205, #103061, .T. ) ;
#21383=VERTEX_POINT ( 'NONE', #92117 ) ;
#21384=EDGE_CURVE ( 'NONE', #107586, #11222, #2811, .T. ) ;
#21385=ORIENTED_EDGE ( 'NONE', *, *, #15977, .T. ) ;
#21387=CARTESIAN_POINT ( 'NONE',  ( -0.4000000000000396572, 12.50000000000000000, 4.330127018922196314 ) ) ;
#21388=CARTESIAN_POINT ( 'NONE',  ( 7.314170287673980475, 2.499999999999874323, 9.688393442490522034 ) ) ;
#21389=CARTESIAN_POINT ( 'NONE',  ( 0.5999999999999560130, 2.500000000000000000, -3.983716857408426293 ) ) ;
#21390=FACE_BOUND ( 'NONE', #38573, .T. ) ;
#21391=DIRECTION ( 'NONE',  ( -0.000000000000000000, 1.000000000000000000, -0.000000000000000000 ) ) ;
#21393=CARTESIAN_POINT ( 'NONE',  ( -10.60000000000000320, 12.50000000000000000, -3.983716857408421852 ) ) ;
#21394=PLANE ( 'NONE',  #85605 ) ;
#21395=EDGE_CURVE ( 'NONE', #83416, #93002, #122038, .T. ) ;
#21396=AXIS2_PLACEMENT_3D ( 'NONE', #122830, #124108, #54089 ) ;
#21397=VECTOR ( 'NONE', #108054, 1000.000000000000000 ) ;
#21398=CARTESIAN_POINT ( 'NONE',  ( 5.849999999999935696, 12.50000000000000000, -7.188010851410854052 ) ) ;
#21399=CIRCLE ( 'NONE', #52705, 0.06509327318403745899 ) ;
#21400=DIRECTION ( 'NONE',  ( 0.000000000000000000, 1.000000000000000000, 0.000000000000000000 ) ) ;
#21401=CARTESIAN_POINT ( 'NONE',  ( -11.44999999999999751, 12.50000000000000000, 6.776507416713035248 ) ) ;
#21402=CIRCLE ( 'NONE', #111269, 0.1000000000000000472 ) ;
#21403=CIRCLE ( 'NONE', #102973, 0.09999999999999982514 ) ;
#21404=CARTESIAN_POINT ( 'NONE',  ( 11.89999999999990798, 2.500000000000000000, 3.983716857408420964 ) ) ;
#21406=ORIENTED_EDGE ( 'NONE', *, *, #112521, .F. ) ;
#21407=VERTEX_POINT ( 'NONE', #51575 ) ;
#21408=ORIENTED_EDGE ( 'NONE', *, *, #50741, .T. ) ;
#21409=ORIENTED_EDGE ( 'NONE', *, *, #117527, .T. ) ;
#21410=CIRCLE ( 'NONE', #38141, 0.1000000000000002554 ) ;
#21411=ORIENTED_EDGE ( 'NONE', *, *, #26814, .F. ) ;
#21413=AXIS2_PLACEMENT_3D ( 'NONE', #107271, #57539, #44484 ) ;
#21414=DIRECTION ( 'NONE',  ( 0.000000000000000000, -0.9999939076577903929, 0.003490651415223739937 ) ) ;
#21415=EDGE_LOOP ( 'NONE', ( #23464, #92906, #42394, #10914 ) ) ;
#21416=FACE_BOUND ( 'NONE', #9701, .T. ) ;
#21417=CONICAL_SURFACE ( 'NONE', #25515, 0.1000000000000000472, 0.003490658503988666988 ) ;
#21418=CARTESIAN_POINT ( 'NONE',  ( 3.949999999999938005, 2.500000000000000000, 6.941600689897073018 ) ) ;
#21419=VERTEX_POINT ( 'NONE', #112426 ) ;
#21420=CARTESIAN_POINT ( 'NONE',  ( 9.599999999999914380, 2.500000000000000000, 3.637306695894644726 ) ) ;
#21421=FACE_OUTER_BOUND ( 'NONE', #71438, .T. ) ;
#21422=FACE_OUTER_BOUND ( 'NONE', #37227, .T. ) ;
#21423=LINE ( 'NONE', #3088, #5711 ) ;
#21424=VERTEX_POINT ( 'NONE', #13556 ) ;
#21425=CARTESIAN_POINT ( 'NONE',  ( 2.699999999999946443, 2.500000000000000000, -4.083716857408426826 ) ) ;
#21426=AXIS2_PLACEMENT_3D ( 'NONE', #8962, #117607, #88822 ) ;
#21427=EDGE_CURVE ( 'NONE', #107613, #119819, #9063, .T. ) ;
#21428=VERTEX_POINT ( 'NONE', #111097 ) ;
#21429=ORIENTED_EDGE ( 'NONE', *, *, #63752, .T. ) ;
#21430=CARTESIAN_POINT ( 'NONE',  ( -10.40000000000000213, 2.500000000000000000, -5.122947341949750211 ) ) ;
#21431=DIRECTION ( 'NONE',  ( 0.000000000000000000, 0.000000000000000000, -1.000000000000000000 ) ) ;
#21432=ORIENTED_EDGE ( 'NONE', *, *, #19447, .T. ) ;
#21433=DIRECTION ( 'NONE',  ( 0.000000000000000000, 0.000000000000000000, -1.000000000000000000 ) ) ;
#21434=CONICAL_SURFACE ( 'NONE', #107103, 0.09999999999999982514, 0.003490658503988666988 ) ;
#21435=VECTOR ( 'NONE', #33517, 1000.000000000000000 ) ;
#21436=FACE_OUTER_BOUND ( 'NONE', #17035, .T. ) ;
#21437=CARTESIAN_POINT ( 'NONE',  ( -6.650000000000014566, 2.500000000000000000, 6.495190528383297135 ) ) ;
#21438=PLANE ( 'NONE',  #93364 ) ;
#21439=CARTESIAN_POINT ( 'NONE',  ( 9.399999999999918643, 2.500000000000000000, -0.3464101615137782364 ) ) ;
#21440=ORIENTED_EDGE ( 'NONE', *, *, #116804, .F. ) ;
#21441=EDGE_CURVE ( 'NONE', #107306, #59034, #105306, .T. ) ;
#21442=CARTESIAN_POINT ( 'NONE',  ( 9.599999999999914380, 12.50000000000000000, -5.022947341949754119 ) ) ;
#21444=ORIENTED_EDGE ( 'NONE', *, *, #74519, .F. ) ;
#21445=DIRECTION ( 'NONE',  ( 0.000000000000000000, 0.000000000000000000, -1.000000000000000000 ) ) ;
#21446=AXIS2_PLACEMENT_3D ( 'NONE', #97141, #72206, #11974 ) ;
#21447=CIRCLE ( 'NONE', #8914, 0.1000000000000002554 ) ;
#21448=EDGE_LOOP ( 'NONE', ( #66724, #15600, #62941, #118164 ) ) ;
#21449=AXIS2_PLACEMENT_3D ( 'NONE', #104269, #53882, #93810 ) ;
#21450=DIRECTION ( 'NONE',  ( -0.000000000000000000, 1.000000000000000000, -0.000000000000000000 ) ) ;
#21451=EDGE_LOOP ( 'NONE', ( #86390, #128742, #63266, #104940 ) ) ;
#21452=CARTESIAN_POINT ( 'NONE',  ( 4.199999999999941558, 2.500000000000000000, -4.430127018922202176 ) ) ;
#21453=DIRECTION ( 'NONE',  ( 0.000000000000000000, 0.000000000000000000, -1.000000000000000000 ) ) ;
#21454=CARTESIAN_POINT ( 'NONE',  ( -7.500000000000013323, 2.500000000000000000, 5.022947341949748790 ) ) ;
#21455=CARTESIAN_POINT ( 'NONE',  ( 5.199999999999937117, 2.500000000000000000, -4.676537180435978769 ) ) ;
#21456=EDGE_CURVE ( 'NONE', #84082, #59400, #61408, .T. ) ;
#21457=DIRECTION ( 'NONE',  ( -0.000000000000000000, 1.000000000000000000, -0.000000000000000000 ) ) ;
#21458=VECTOR ( 'NONE', #58269, 1000.000000000000000 ) ;
#21461=CONICAL_SURFACE ( 'NONE', #94605, 0.1000000000000002554, 0.003490658503988666988 ) ;
#21462=ORIENTED_EDGE ( 'NONE', *, *, #26484, .T. ) ;
#21463=FACE_OUTER_BOUND ( 'NONE', #73460, .T. ) ;
#21464=CARTESIAN_POINT ( 'NONE',  ( 7.299999999999926104, 2.500000000000000000, 4.676537180435972552 ) ) ;
#21465=VECTOR ( 'NONE', #87627, 1000.000000000000000 ) ;
#21466=AXIS2_PLACEMENT_3D ( 'NONE', #119201, #77984, #57714 ) ;
#21467=CONICAL_SURFACE ( 'NONE', #523, 0.09999999999999982514, 0.003490658503988666988 ) ;
#21468=DIRECTION ( 'NONE',  ( 0.000000000000000000, -0.000000000000000000, 1.000000000000000000 ) ) ;
#21469=ORIENTED_EDGE ( 'NONE', *, *, #95197, .T. ) ;
#21470=EDGE_LOOP ( 'NONE', ( #37722, #39244 ) ) ;
#21471=ORIENTED_EDGE ( 'NONE', *, *, #11463, .F. ) ;
#21472=CARTESIAN_POINT ( 'NONE',  ( -1.250000000000037970, 2.500000000000000000, 2.757883832488649656 ) ) ;
#21473=VECTOR ( 'NONE', #55550, 1000.000000000000000 ) ;
#21474=ORIENTED_EDGE ( 'NONE', *, *, #5384, .T. ) ;
#21475=DIRECTION ( 'NONE',  ( 0.000000000000000000, -0.000000000000000000, 1.000000000000000000 ) ) ;
#21476=DIRECTION ( 'NONE',  ( 0.000000000000000000, -0.000000000000000000, 1.000000000000000000 ) ) ;
#21477=FACE_OUTER_BOUND ( 'NONE', #13006, .T. ) ;
#21478=CARTESIAN_POINT ( 'NONE',  ( 12.89999999999989910, 2.500000000000000000, -0.5928203230275542746 ) ) ;
#21479=LINE ( 'NONE', #63339, #75829 ) ;
#21480=CARTESIAN_POINT ( 'NONE',  ( 13.34999999999989662, 12.50000000000000000, -1.537336459617587581 ) ) ;
#21481=DIRECTION ( 'NONE',  ( -4.274815082592931898E-19, -0.9999939076577903929, -0.003490651415223739937 ) ) ;
#21482=DIRECTION ( 'NONE',  ( -0.000000000000000000, -1.000000000000000000, -0.000000000000000000 ) ) ;
#21483=ORIENTED_EDGE ( 'NONE', *, *, #128642, .T. ) ;
#21484=ADVANCED_FACE ( 'NONE', ( #1801 ), #82234, .T. ) ;
#21485=CARTESIAN_POINT ( 'NONE',  ( -13.29999999999999005, 2.500000000000000000, -4.230127018922199333 ) ) ;
#21486=DIRECTION ( 'NONE',  ( -0.000000000000000000, -1.000000000000000000, -0.000000000000000000 ) ) ;
#21487=ORIENTED_EDGE ( 'NONE', *, *, #71553, .T. ) ;
#21488=ORIENTED_EDGE ( 'NONE', *, *, #121115, .F. ) ;
#21489=CIRCLE ( 'NONE', #61204, 0.06509327318403745899 ) ;
#21490=ADVANCED_FACE ( 'NONE', ( #25975 ), #6988, .T. ) ;
#21493=DIRECTION ( 'NONE',  ( 0.000000000000000000, 0.000000000000000000, 1.000000000000000000 ) ) ;
#21494=ADVANCED_FACE ( 'NONE', ( #85531 ), #90631, .T. ) ;
#21495=CARTESIAN_POINT ( 'NONE',  ( -12.69999999999999396, 12.50000000000000000, -3.983716857408423628 ) ) ;
#21496=CARTESIAN_POINT ( 'NONE',  ( 13.74999999999993072, 2.500000000000000000, -2.165063509461101710 ) ) ;
#21497=CARTESIAN_POINT ( 'NONE',  ( -13.74999999999995381, 12.50000000000000000, -2.230156782645137170 ) ) ;
#21498=AXIS2_PLACEMENT_3D ( 'NONE', #1598, #18670, #71003 ) ;
#21499=DIRECTION ( 'NONE',  ( -0.000000000000000000, -1.000000000000000000, -0.000000000000000000 ) ) ;
#21500=DIRECTION ( 'NONE',  ( -4.274815082592931898E-19, -0.9999939076577903929, -0.003490651415223739937 ) ) ;
#21501=AXIS2_PLACEMENT_3D ( 'NONE', #82480, #12422, #93578 ) ;
#21502=ADVANCED_FACE ( 'NONE', ( #105164 ), #115668, .T. ) ;
#21503=VECTOR ( 'NONE', #33111, 1000.000000000000000 ) ;
#21504=EDGE_CURVE ( 'NONE', #49723, #58972, #42539, .T. ) ;
#21505=ADVANCED_FACE ( 'NONE', ( #5020 ), #25792, .T. ) ;
#21506=DIRECTION ( 'NONE',  ( 0.000000000000000000, 1.000000000000000000, 0.000000000000000000 ) ) ;
#21507=ORIENTED_EDGE ( 'NONE', *, *, #116766, .T. ) ;
#21508=CIRCLE ( 'NONE', #652, 0.06509327318403745899 ) ;
#21509=VERTEX_POINT ( 'NONE', #125452 ) ;
#21510=VECTOR ( 'NONE', #44868, 1000.000000000000000 ) ;
#21511=ADVANCED_FACE ( 'NONE', ( #6298 ), #116269, .T. ) ;
#21512=ORIENTED_EDGE ( 'NONE', *, *, #32590, .F. ) ;
#21513=AXIS2_PLACEMENT_3D ( 'NONE', #37249, #82644, #105971 ) ;
#21514=CIRCLE ( 'NONE', #121958, 0.09999999999999982514 ) ;
#21516=CARTESIAN_POINT ( 'NONE',  ( -8.150000000000014566, 12.50000000000000000, -6.841600689897073373 ) ) ;
#21517=CARTESIAN_POINT ( 'NONE',  ( 11.24999999999990941, 2.500000000000000000, 7.188010851410848723 ) ) ;
#21518=ADVANCED_FACE ( 'NONE', ( #86815 ), #80173, .T. ) ;
#21519=ORIENTED_EDGE ( 'NONE', *, *, #52733, .T. ) ;
#21520=CARTESIAN_POINT ( 'NONE',  ( 12.69999999999990337, 2.500000000000000000, -4.576537180435978236 ) ) ;
#21521=CARTESIAN_POINT ( 'NONE',  ( -7.900000000000014566, 12.50000000000000000, -0.6277270498435166823 ) ) ;
#21522=LINE ( 'NONE', #10405, #49370 ) ;
#21525=DIRECTION ( 'NONE',  ( 0.000000000000000000, 0.000000000000000000, 1.000000000000000000 ) ) ;
#21526=CONICAL_SURFACE ( 'NONE', #19358, 0.1000000000000002554, 0.003490658503988666988 ) ;
#21527=CARTESIAN_POINT ( 'NONE',  ( 6.649999999999931077, 2.500000000000000000, -6.495190528383302464 ) ) ;
#21528=ORIENTED_EDGE ( 'NONE', *, *, #45848, .F. ) ;
#21530=EDGE_LOOP ( 'NONE', ( #40027, #9508 ) ) ;
#21531=ORIENTED_EDGE ( 'NONE', *, *, #22675, .T. ) ;
#21532=CARTESIAN_POINT ( 'NONE',  ( -2.100000000000034284, 12.50000000000000000, -4.330127018922201643 ) ) ;
#21533=CARTESIAN_POINT ( 'NONE',  ( -11.89999999999999680, 12.50000000000000000, -0.2813168883297367806 ) ) ;
#21534=AXIS2_PLACEMENT_3D ( 'NONE', #64347, #62434, #52592 ) ;
#21535=CARTESIAN_POINT ( 'NONE',  ( -14.99999999999994671, 2.500000000000000000, 0.1000000000000000056 ) ) ;
#21536=VECTOR ( 'NONE', #99178, 1000.000000000000000 ) ;
#21538=CARTESIAN_POINT ( 'NONE',  ( -1.050000000000038680, 2.500000000000000000, 6.841600689897072485 ) ) ;
#21539=ORIENTED_EDGE ( 'NONE', *, *, #111762, .F. ) ;
#21540=LINE ( 'NONE', #70637, #3538 ) ;
#21541=DIRECTION ( 'NONE',  ( 0.000000000000000000, 1.000000000000000000, 0.000000000000000000 ) ) ;
#21542=CARTESIAN_POINT ( 'NONE',  ( -5.650000000000023448, 2.500000000000000000, -6.148780366869526226 ) ) ;
#21543=DIRECTION ( 'NONE',  ( 0.000000000000000000, -0.000000000000000000, 1.000000000000000000 ) ) ;
#21544=CIRCLE ( 'NONE', #6840, 0.06509327318403745899 ) ;
#21545=CONICAL_SURFACE ( 'NONE', #125986, 0.09999999999999982514, 0.003490658503988666988 ) ;
#21546=AXIS2_PLACEMENT_3D ( 'NONE', #7256, #77305, #120452 ) ;
#21547=ORIENTED_EDGE ( 'NONE', *, *, #2264, .T. ) ;
#21548=VECTOR ( 'NONE', #115349, 1000.000000000000000 ) ;
#21550=VERTEX_POINT ( 'NONE', #5662 ) ;
#21551=VERTEX_POINT ( 'NONE', #14826 ) ;
#21552=CARTESIAN_POINT ( 'NONE',  ( -6.650000000000014566, 12.50000000000000000, 6.560283801567334372 ) ) ;
#21553=DIRECTION ( 'NONE',  ( 0.000000000000000000, 0.000000000000000000, -1.000000000000000000 ) ) ;
#21554=FACE_BOUND ( 'NONE', #102693, .T. ) ;
#21555=DIRECTION ( 'NONE',  ( 0.000000000000000000, 0.000000000000000000, 1.000000000000000000 ) ) ;
#21556=CONICAL_SURFACE ( 'NONE', #94704, 0.09999999999999982514, 0.003490658503988666988 ) ;
#21557=DIRECTION ( 'NONE',  ( -0.000000000000000000, 1.000000000000000000, -0.000000000000000000 ) ) ;
#21558=DIRECTION ( 'NONE',  ( 0.000000000000000000, 1.000000000000000000, 0.000000000000000000 ) ) ;
#21559=ADVANCED_FACE ( 'NONE', ( #24684 ), #64599, .T. ) ;
#21560=AXIS2_PLACEMENT_3D ( 'NONE', #12922, #101980, #31957 ) ;
#21561=VECTOR ( 'NONE', #63188, 1000.000000000000000 ) ;
#21562=AXIS2_PLACEMENT_3D ( 'NONE', #39193, #79734, #86972 ) ;
#21563=DIRECTION ( 'NONE',  ( 0.000000000000000000, 1.000000000000000000, 0.000000000000000000 ) ) ;
#21564=DIRECTION ( 'NONE',  ( 0.000000000000000000, 0.000000000000000000, 1.000000000000000000 ) ) ;
#21565=VECTOR ( 'NONE', #43026, 1000.000000000000000 ) ;
#21566=CARTESIAN_POINT ( 'NONE',  ( -9.150000000000009237, 12.50000000000000000, -1.472243186433550122 ) ) ;
#21567=EDGE_LOOP ( 'NONE', ( #98839, #100226, #90229, #16865 ) ) ;
#21568=DIRECTION ( 'NONE',  ( -0.000000000000000000, -1.000000000000000000, -0.000000000000000000 ) ) ;
#21569=LINE ( 'NONE', #121690, #64279 ) ;
#21570=CIRCLE ( 'NONE', #69390, 0.06509327318403745899 ) ;
#21571=VERTEX_POINT ( 'NONE', #126091 ) ;
#21572=ORIENTED_EDGE ( 'NONE', *, *, #77750, .T. ) ;
#21573=CARTESIAN_POINT ( 'NONE',  ( -2.900000000000029221, 12.50000000000000000, -5.022947341949754119 ) ) ;
#21574=DIRECTION ( 'NONE',  ( 0.000000000000000000, 1.000000000000000000, 0.000000000000000000 ) ) ;
#21575=FACE_BOUND ( 'NONE', #59744, .T. ) ;
#21576=CARTESIAN_POINT ( 'NONE',  ( 6.249999999999932498, 2.500000000000000000, -5.802370205355749988 ) ) ;
#21577=AXIS2_PLACEMENT_3D ( 'NONE', #80414, #29384, #90199 ) ;
#21578=EDGE_LOOP ( 'NONE', ( #59106, #67275 ) ) ;
#21579=CARTESIAN_POINT ( 'NONE',  ( 4.399999999999939071, 2.500000000000000000, -0.3464101615137782364 ) ) ;
#21580=CIRCLE ( 'NONE', #73899, 0.1000000000000002554 ) ;
#21581=DIRECTION ( 'NONE',  ( -0.000000000000000000, -1.000000000000000000, -0.000000000000000000 ) ) ;
#21582=EDGE_LOOP ( 'NONE', ( #69399, #18895, #2034, #56270 ) ) ;
#21583=FACE_OUTER_BOUND ( 'NONE', #87543, .T. ) ;
#21584=FACE_OUTER_BOUND ( 'NONE', #88625, .T. ) ;
#21585=ADVANCED_FACE ( 'NONE', ( #56689 ), #30013, .T. ) ;
#21587=CONICAL_SURFACE ( 'NONE', #67534, 0.1000000000000002554, 0.003490658503988666988 ) ;
#21588=AXIS2_PLACEMENT_3D ( 'NONE', #109841, #68614, #50278 ) ;
#21589=AXIS2_PLACEMENT_3D ( 'NONE', #84768, #116147, #124697 ) ;
#21590=DIRECTION ( 'NONE',  ( -4.274815082592931898E-19, -0.9999939076577903929, -0.003490651415223739937 ) ) ;
#21591=DIRECTION ( 'NONE',  ( -0.000000000000000000, 1.000000000000000000, -0.000000000000000000 ) ) ;
#21593=AXIS2_PLACEMENT_3D ( 'NONE', #104732, #75930, #115183 ) ;
#21594=AXIS2_PLACEMENT_3D ( 'NONE', #48674, #10035, #855 ) ;
#21595=ORIENTED_EDGE ( 'NONE', *, *, #58363, .T. ) ;
#21596=DIRECTION ( 'NONE',  ( -0.000000000000000000, 1.000000000000000000, -0.000000000000000000 ) ) ;
#21597=PLANE ( 'NONE',  #22540 ) ;
#21598=CARTESIAN_POINT ( 'NONE',  ( -12.49999999999995914, 2.500000000000000000, 1.843143693225357538E-15 ) ) ;
#21599=AXIS2_PLACEMENT_3D ( 'NONE', #81031, #61395, #11636 ) ;
#21600=AXIS2_PLACEMENT_3D ( 'NONE', #94401, #113411, #45329 ) ;
#21601=ORIENTED_EDGE ( 'NONE', *, *, #95960, .F. ) ;
#21602=EDGE_CURVE ( 'NONE', #99945, #46684, #57188, .T. ) ;
#21603=EDGE_LOOP ( 'NONE', ( #116989, #11284, #19680, #42295 ) ) ;
#21605=CARTESIAN_POINT ( 'NONE',  ( -6.050000000000017586, 2.500000000000000000, 6.248780366869520542 ) ) ;
#21606=CIRCLE ( 'NONE', #32087, 0.1000000000000002554 ) ;
#21607=ORIENTED_EDGE ( 'NONE', *, *, #122559, .T. ) ;
#21608=PLANE ( 'NONE',  #15674 ) ;
#21609=CARTESIAN_POINT ( 'NONE',  ( 9.149999999999920419, 2.500000000000000000, 2.957883832488649389 ) ) ;
#21610=DIRECTION ( 'NONE',  ( 0.000000000000000000, 0.000000000000000000, -1.000000000000000000 ) ) ;
#21611=VERTEX_POINT ( 'NONE', #37088 ) ;
#21612=ADVANCED_FACE ( 'NONE', ( #106458 ), #17461, .T. ) ;
#21613=CARTESIAN_POINT ( 'NONE',  ( 2.899999999999944844, 2.500000000000000000, 5.022947341949748790 ) ) ;
#21614=CARTESIAN_POINT ( 'NONE',  ( -5.850000000000021849, 12.50000000000000000, -2.857883832488653741 ) ) ;
#21615=DIRECTION ( 'NONE',  ( 0.000000000000000000, 0.000000000000000000, 1.000000000000000000 ) ) ;
#21616=LINE ( 'NONE', #81183, #108210 ) ;
#21617=PLANE ( 'NONE',  #67399 ) ;
#21618=EDGE_CURVE ( 'NONE', #78911, #48128, #126143, .T. ) ;
#21619=DIRECTION ( 'NONE',  ( 0.000000000000000000, -0.000000000000000000, 1.000000000000000000 ) ) ;
#21620=CIRCLE ( 'NONE', #78048, 0.06509327318403741736 ) ;
#21621=ORIENTED_EDGE ( 'NONE', *, *, #97283, .T. ) ;
#21622=EDGE_LOOP ( 'NONE', ( #120827, #34843, #108432, #4365 ) ) ;
#21623=DIRECTION ( 'NONE',  ( -0.000000000000000000, 1.000000000000000000, -0.000000000000000000 ) ) ;
#21624=EDGE_LOOP ( 'NONE', ( #9245, #12325 ) ) ;
#21625=LINE ( 'NONE', #70083, #61918 ) ;
#21626=ORIENTED_EDGE ( 'NONE', *, *, #90922, .F. ) ;
#21627=EDGE_LOOP ( 'NONE', ( #116586, #98430, #58807, #87717 ) ) ;
#21628=VERTEX_POINT ( 'NONE', #78953 ) ;
#21629=CARTESIAN_POINT ( 'NONE',  ( -11.89999999999999680, 2.500000000000000000, -4.676537180435976104 ) ) ;
#21630=CONICAL_SURFACE ( 'NONE', #17397, 0.09999999999999982514, 0.003490658503988666988 ) ;
#21631=AXIS2_PLACEMENT_3D ( 'NONE', #44109, #84024, #55858 ) ;
#21632=CARTESIAN_POINT ( 'NONE',  ( 4.349999999999938360, 2.500000000000000000, 1.818653347947321475 ) ) ;
#21633=AXIS2_PLACEMENT_3D ( 'NONE', #118140, #129281, #28482 ) ;
#21634=CARTESIAN_POINT ( 'NONE',  ( 5.599999999999933031, 2.500000000000000000, 0.3464101615137735735 ) ) ;
#21636=DIRECTION ( 'NONE',  ( 0.000000000000000000, 1.000000000000000000, 0.000000000000000000 ) ) ;
#21637=FACE_OUTER_BOUND ( 'NONE', #21255, .T. ) ;
#21638=DIRECTION ( 'NONE',  ( 0.000000000000000000, -0.9999939076577903929, 0.003490651415223739937 ) ) ;
#21639=DIRECTION ( 'NONE',  ( -4.274815082592931898E-19, -0.9999939076577903929, -0.003490651415223739937 ) ) ;
#21640=FACE_OUTER_BOUND ( 'NONE', #24442, .T. ) ;
#21641=CONICAL_SURFACE ( 'NONE', #115617, 0.1000000000000002554, 0.003490658503988666988 ) ;
#21643=VECTOR ( 'NONE', #54757, 1000.000000000000000 ) ;
#21644=VERTEX_POINT ( 'NONE', #119494 ) ;
#21645=AXIS2_PLACEMENT_3D ( 'NONE', #41979, #34093, #113938 ) ;
#21646=EDGE_CURVE ( 'NONE', #51736, #111655, #4931, .T. ) ;
#21647=DIRECTION ( 'NONE',  ( 0.000000000000000000, 1.000000000000000000, 0.000000000000000000 ) ) ;
#21648=EDGE_LOOP ( 'NONE', ( #77586, #22706, #119675, #56170 ) ) ;
#21649=EDGE_LOOP ( 'NONE', ( #59104, #357, #77097, #119739 ) ) ;
#21650=DIRECTION ( 'NONE',  ( -0.000000000000000000, -1.000000000000000000, -0.000000000000000000 ) ) ;
#21651=DIRECTION ( 'NONE',  ( 0.000000000000000000, -0.9999939076577903929, 0.003490651415223739937 ) ) ;
#21652=CIRCLE ( 'NONE', #107612, 0.1000000000000000472 ) ;
#21653=DIRECTION ( 'NONE',  ( 0.000000000000000000, 0.000000000000000000, 1.000000000000000000 ) ) ;
#21654=EDGE_CURVE ( 'NONE', #108166, #82548, #71869, .T. ) ;
#21655=DIRECTION ( 'NONE',  ( 0.000000000000000000, 0.000000000000000000, 1.000000000000000000 ) ) ;
#21656=CARTESIAN_POINT ( 'NONE',  ( 15.39999999999989200, 2.500000000000000000, -0.5928203230275542746 ) ) ;
#21657=AXIS2_PLACEMENT_3D ( 'NONE', #120105, #30453, #70352 ) ;
#21658=DIRECTION ( 'NONE',  ( 0.000000000000000000, 0.000000000000000000, 1.000000000000000000 ) ) ;
#21659=CONICAL_SURFACE ( 'NONE', #34188, 0.09999999999999982514, 0.003490658503988666988 ) ;
#21660=AXIS2_PLACEMENT_3D ( 'NONE', #37089, #127399, #118214 ) ;
#21661=LINE ( 'NONE', #89747, #42551 ) ;
#21662=ORIENTED_EDGE ( 'NONE', *, *, #119862, .T. ) ;
#21663=EDGE_CURVE ( 'NONE', #24371, #24257, #119883, .T. ) ;
#21664=CIRCLE ( 'NONE', #73884, 0.1000000000000002554 ) ;
#21665=EDGE_CURVE ( 'NONE', #113481, #90527, #15397, .T. ) ;
#21666=EDGE_CURVE ( 'NONE', #67886, #14684, #124080, .T. ) ;
#21667=AXIS2_PLACEMENT_3D ( 'NONE', #107539, #36874, #97710 ) ;
#21668=ORIENTED_EDGE ( 'NONE', *, *, #29629, .T. ) ;
#21669=ORIENTED_EDGE ( 'NONE', *, *, #14564, .T. ) ;
#21670=ADVANCED_FACE ( 'NONE', ( #118856 ), #78129, .T. ) ;
#21671=ORIENTED_EDGE ( 'NONE', *, *, #107475, .T. ) ;
#21672=ORIENTED_EDGE ( 'NONE', *, *, #47397, .F. ) ;
#21673=DIRECTION ( 'NONE',  ( -0.000000000000000000, -1.000000000000000000, -0.000000000000000000 ) ) ;
#21674=FACE_OUTER_BOUND ( 'NONE', #52841, .T. ) ;
#21675=ADVANCED_FACE ( 'NONE', ( #40315 ), #111562, .T. ) ;
#21676=ADVANCED_FACE ( 'NONE', ( #90023 ), #40584, .T. ) ;
#21677=LINE ( 'NONE', #20385, #111485 ) ;
#21678=CARTESIAN_POINT ( 'NONE',  ( -0.6000000000000388356, 2.500000000000000000, 4.776537180435972196 ) ) ;
#21679=DIRECTION ( 'NONE',  ( 0.000000000000000000, -0.000000000000000000, 1.000000000000000000 ) ) ;
#21680=ORIENTED_EDGE ( 'NONE', *, *, #11314, .T. ) ;
#21681=CARTESIAN_POINT ( 'NONE',  ( -14.39999999999998614, 2.500000000000000000, -0.3464101615137760715 ) ) ;
#21682=DIRECTION ( 'NONE',  ( 0.000000000000000000, 0.000000000000000000, 1.000000000000000000 ) ) ;
#21683=AXIS2_PLACEMENT_3D ( 'NONE', #25330, #36479, #96637 ) ;
#21684=AXIS2_PLACEMENT_3D ( 'NONE', #63460, #103382, #75836 ) ;
#21685=CARTESIAN_POINT ( 'NONE',  ( -5.850000000000022737, 2.500000000000000000, -2.165063509461101710 ) ) ;
#21686=DIRECTION ( 'NONE',  ( 0.000000000000000000, 1.000000000000000000, 0.000000000000000000 ) ) ;
#21687=DIRECTION ( 'NONE',  ( 0.000000000000000000, 0.000000000000000000, 1.000000000000000000 ) ) ;
#21688=ORIENTED_EDGE ( 'NONE', *, *, #77901, .T. ) ;
#21689=CONICAL_SURFACE ( 'NONE', #107350, 0.1000000000000002554, 0.003490658503988666988 ) ;
#21690=CIRCLE ( 'NONE', #61405, 0.06509327318403745899 ) ;
#21691=ORIENTED_EDGE ( 'NONE', *, *, #67572, .F. ) ;
#21692=ORIENTED_EDGE ( 'NONE', *, *, #17914, .T. ) ;
#21693=AXIS2_PLACEMENT_3D ( 'NONE', #34890, #96346, #13922 ) ;
#21694=DIRECTION ( 'NONE',  ( 0.000000000000000000, 1.000000000000000000, 0.000000000000000000 ) ) ;
#21695=ORIENTED_EDGE ( 'NONE', *, *, #24774, .T. ) ;
#21696=CARTESIAN_POINT ( 'NONE',  ( 9.149999999999918643, 2.500000000000000000, -6.495190528383302464 ) ) ;
#21697=DIRECTION ( 'NONE',  ( -0.000000000000000000, 1.000000000000000000, -0.000000000000000000 ) ) ;
#21698=AXIS2_PLACEMENT_3D ( 'NONE', #34749, #36018, #95583 ) ;
#21699=CONICAL_SURFACE ( 'NONE', #32078, 0.09999999999999982514, 0.003490658503988666988 ) ;
#21700=VECTOR ( 'NONE', #127197, 1000.000000000000000 ) ;
#21701=CIRCLE ( 'NONE', #94851, 0.06509327318403743123 ) ;
#21702=EDGE_LOOP ( 'NONE', ( #583, #54217, #24754, #91011 ) ) ;
#21703=CARTESIAN_POINT ( 'NONE',  ( -0.6500000000000389910, 12.50000000000000000, -1.818653347947326138 ) ) ;
#21704=CARTESIAN_POINT ( 'NONE',  ( 7.499999999999927169, 12.50000000000000000, 3.637306695894644726 ) ) ;
#21705=FACE_OUTER_BOUND ( 'NONE', #39190, .T. ) ;
#21706=FACE_OUTER_BOUND ( 'NONE', #101436, .T. ) ;
#21707=DIRECTION ( 'NONE',  ( 0.000000000000000000, 1.000000000000000000, 0.000000000000000000 ) ) ;
#21708=VERTEX_POINT ( 'NONE', #109691 ) ;
#21709=ORIENTED_EDGE ( 'NONE', *, *, #102018, .T. ) ;
#21710=FACE_OUTER_BOUND ( 'NONE', #78756, .T. ) ;
#21711=DIRECTION ( 'NONE',  ( 0.000000000000000000, 0.000000000000000000, 1.000000000000000000 ) ) ;
#21712=DIRECTION ( 'NONE',  ( 0.000000000000000000, 0.000000000000000000, 1.000000000000000000 ) ) ;
#21713=CARTESIAN_POINT ( 'NONE',  ( 0.4499999999999573785, 2.500000000000000000, -6.495190528383302464 ) ) ;
#21714=EDGE_CURVE ( 'NONE', #113119, #90074, #69806, .T. ) ;
#21715=EDGE_LOOP ( 'NONE', ( #124464, #29054, #56279, #47572 ) ) ;
#21716=ORIENTED_EDGE ( 'NONE', *, *, #16450, .F. ) ;
#21717=CARTESIAN_POINT ( 'NONE',  ( 11.44999999999990870, 2.500000000000000000, 6.841600689897072485 ) ) ;
#21718=CARTESIAN_POINT ( 'NONE',  ( -11.69999999999999929, 2.500000000000000000, 1.734723475976807094E-15 ) ) ;
#21719=CARTESIAN_POINT ( 'NONE',  ( 0.6499999999999566125, 12.50000000000000000, -6.148780366869526226 ) ) ;
#21720=CIRCLE ( 'NONE', #88309, 0.06509327318403745899 ) ;
#21721=CARTESIAN_POINT ( 'NONE',  ( 12.69999999999990159, 2.500000000000000000, -4.083716857408426826 ) ) ;
#21722=ORIENTED_EDGE ( 'NONE', *, *, #41881, .F. ) ;
#21723=CONICAL_SURFACE ( 'NONE', #109452, 0.09999999999999982514, 0.003490658503988666988 ) ;
#21724=CONICAL_SURFACE ( 'NONE', #67774, 0.09999999999999982514, 0.003490658503988666988 ) ;
#21725=FACE_OUTER_BOUND ( 'NONE', #11986, .T. ) ;
#21726=CARTESIAN_POINT ( 'NONE',  ( 3.349999999999941913, 2.500000000000000000, 5.802370205355744659 ) ) ;
#21727=ORIENTED_EDGE ( 'NONE', *, *, #70151, .T. ) ;
#21728=CARTESIAN_POINT ( 'NONE',  ( 6.449999999999931788, 2.500000000000000000, -6.148780366869526226 ) ) ;
#21730=ORIENTED_EDGE ( 'NONE', *, *, #66679, .T. ) ;
#21731=VECTOR ( 'NONE', #10839, 1000.000000000000000 ) ;
#21732=DIRECTION ( 'NONE',  ( 0.000000000000000000, 1.000000000000000000, 0.000000000000000000 ) ) ;
#21733=CIRCLE ( 'NONE', #13305, 0.09999999999999982514 ) ;
#21734=ORIENTED_EDGE ( 'NONE', *, *, #52932, .T. ) ;
#21735=AXIS2_PLACEMENT_3D ( 'NONE', #42976, #25878, #53417 ) ;
#21736=ORIENTED_EDGE ( 'NONE', *, *, #110052, .F. ) ;
#21737=CARTESIAN_POINT ( 'NONE',  ( -10.00000000000000533, 2.500000000000000000, 0.6928203230275494784 ) ) ;
#21739=EDGE_LOOP ( 'NONE', ( #19311, #108600 ) ) ;
#21740=ORIENTED_EDGE ( 'NONE', *, *, #9213, .F. ) ;
#21741=AXIS2_PLACEMENT_3D ( 'NONE', #109002, #68440, #18049 ) ;
#21742=DIRECTION ( 'NONE',  ( -4.274815082592931898E-19, -0.9999939076577903929, -0.003490651415223739937 ) ) ;
#21743=DIRECTION ( 'NONE',  ( 0.000000000000000000, -0.000000000000000000, 1.000000000000000000 ) ) ;
#21744=ORIENTED_EDGE ( 'NONE', *, *, #8200, .F. ) ;
#21745=CARTESIAN_POINT ( 'NONE',  ( 1.249999999999952038, 12.50000000000000000, -1.407149913249512663 ) ) ;
#21747=CARTESIAN_POINT ( 'NONE',  ( 0.7999999999999548583, 2.500000000000000000, 4.430127018922196847 ) ) ;
#21748=VECTOR ( 'NONE', #67583, 1000.000000000000000 ) ;
#21749=CARTESIAN_POINT ( 'NONE',  ( -2.900000000000029221, 2.500000000000000000, -5.122947341949753763 ) ) ;
#21750=FACE_OUTER_BOUND ( 'NONE', #95351, .T. ) ;
#21751=CARTESIAN_POINT ( 'NONE',  ( 8.149999999999920419, 12.50000000000000000, 6.776507416713035248 ) ) ;
#21752=CIRCLE ( 'NONE', #48949, 0.09999999999999982514 ) ;
#21753=FACE_OUTER_BOUND ( 'NONE', #17128, .T. ) ;
#21754=AXIS2_PLACEMENT_3D ( 'NONE', #69864, #89500, #109786 ) ;
#21755=EDGE_CURVE ( 'NONE', #90522, #77475, #65675, .T. ) ;
#21756=ORIENTED_EDGE ( 'NONE', *, *, #50319, .F. ) ;
#21757=VERTEX_POINT ( 'NONE', #7607 ) ;
#21758=CARTESIAN_POINT ( 'NONE',  ( -9.350000000000006750, 12.50000000000000000, -2.511473670974877948 ) ) ;
#21759=ORIENTED_EDGE ( 'NONE', *, *, #47965, .F. ) ;
#21760=CARTESIAN_POINT ( 'NONE',  ( 11.04999999999990656, 2.500000000000000000, -6.148780366869526226 ) ) ;
#21761=FACE_OUTER_BOUND ( 'NONE', #114281, .T. ) ;
#21762=DIRECTION ( 'NONE',  ( 0.000000000000000000, 0.000000000000000000, -1.000000000000000000 ) ) ;
#21763=ORIENTED_EDGE ( 'NONE', *, *, #115422, .T. ) ;
#21764=ORIENTED_EDGE ( 'NONE', *, *, #30403, .F. ) ;
#21765=ADVANCED_FACE ( 'NONE', ( #99875 ), #353, .T. ) ;
#21766=FACE_BOUND ( 'NONE', #39678, .T. ) ;
#21767=ORIENTED_EDGE ( 'NONE', *, *, #38743, .F. ) ;
#21768=ADVANCED_FACE ( 'NONE', ( #127398 ), #49499, .T. ) ;
#21769=FACE_OUTER_BOUND ( 'NONE', #110643, .T. ) ;
#21770=FACE_OUTER_BOUND ( 'NONE', #37755, .T. ) ;
#21771=CARTESIAN_POINT ( 'NONE',  ( 8.949999999999919353, 2.500000000000000000, -6.248780366869526759 ) ) ;
#21773=CARTESIAN_POINT ( 'NONE',  ( -5.850000000000018296, 2.500000000000000000, 5.702370205355745014 ) ) ;
#21774=CARTESIAN_POINT ( 'NONE',  ( -10.65000000000000213, 2.500000000000000000, 6.841600689897072485 ) ) ;
#21775=EDGE_CURVE ( 'NONE', #105608, #86126, #80233, .T. ) ;
#21776=CONICAL_SURFACE ( 'NONE', #105387, 0.1000000000000002554, 0.003490658503988666988 ) ;
#21777=DIRECTION ( 'NONE',  ( 0.000000000000000000, 0.000000000000000000, 1.000000000000000000 ) ) ;
#21778=EDGE_CURVE ( 'NONE', #82940, #99080, #58018, .T. ) ;
#21779=CARTESIAN_POINT ( 'NONE',  ( -2.900000000000030109, 12.50000000000000000, 0.6928203230275494784 ) ) ;
#21780=CONICAL_SURFACE ( 'NONE', #109602, 0.1000000000000002554, 0.003490658503988666988 ) ;
#21781=CONICAL_SURFACE ( 'NONE', #38512, 0.09999999999999982514, 0.003490658503988666988 ) ;
#21782=DIRECTION ( 'NONE',  ( 0.000000000000000000, -0.9999939076577903929, 0.003490651415223739937 ) ) ;
#21783=CARTESIAN_POINT ( 'NONE',  ( 4.399999999999939071, 12.50000000000000000, -0.2813168883297408329 ) ) ;
#21784=EDGE_CURVE ( 'NONE', #103084, #47024, #5033, .T. ) ;
#21785=LINE ( 'NONE', #62981, #116118 ) ;
#21786=AXIS2_PLACEMENT_3D ( 'NONE', #72270, #64990, #104294 ) ;
#21787=CIRCLE ( 'NONE', #69801, 0.06509327318403745899 ) ;
#21788=EDGE_LOOP ( 'NONE', ( #38789, #96304, #104229, #81836 ) ) ;
#21789=ORIENTED_EDGE ( 'NONE', *, *, #91262, .F. ) ;
#21790=EDGE_LOOP ( 'NONE', ( #78838, #77133, #5114, #330 ) ) ;
#21791=AXIS2_PLACEMENT_3D ( 'NONE', #69004, #39586, #48741 ) ;
#21792=EDGE_LOOP ( 'NONE', ( #80445, #77387, #86813, #44809 ) ) ;
#21793=CARTESIAN_POINT ( 'NONE',  ( -3.100000000000028955, 2.500000000000000000, 4.676537180435972552 ) ) ;
#21794=AXIS2_PLACEMENT_3D ( 'NONE', #122730, #70407, #41611 ) ;
#21795=DIRECTION ( 'NONE',  ( -0.000000000000000000, -1.000000000000000000, -0.000000000000000000 ) ) ;
#21796=ORIENTED_EDGE ( 'NONE', *, *, #100693, .T. ) ;
#21797=ORIENTED_EDGE ( 'NONE', *, *, #114001, .T. ) ;
#21798=ORIENTED_EDGE ( 'NONE', *, *, #88887, .F. ) ;
#21799=DIRECTION ( 'NONE',  ( 0.000000000000000000, 1.000000000000000000, 0.000000000000000000 ) ) ;
#21800=AXIS2_PLACEMENT_3D ( 'NONE', #8469, #58881, #117771 ) ;
#21801=CONICAL_SURFACE ( 'NONE', #48897, 0.1000000000000002554, 0.003490658503988666988 ) ;
#21803=DIRECTION ( 'NONE',  ( -0.000000000000000000, 1.000000000000000000, -0.000000000000000000 ) ) ;
#21804=DIRECTION ( 'NONE',  ( 0.000000000000000000, 0.000000000000000000, 1.000000000000000000 ) ) ;
#21805=CARTESIAN_POINT ( 'NONE',  ( 12.09999999999990550, 2.500000000000000000, 4.922947341949748257 ) ) ;
#21806=CARTESIAN_POINT ( 'NONE',  ( -8.350000000000013856, 12.50000000000000000, 2.165063509461097713 ) ) ;
#21807=DIRECTION ( 'NONE',  ( 0.000000000000000000, 1.000000000000000000, 0.000000000000000000 ) ) ;
#21808=VERTEX_POINT ( 'NONE', #20025 ) ;
#21811=ORIENTED_EDGE ( 'NONE', *, *, #6821, .T. ) ;
#21812=ORIENTED_EDGE ( 'NONE', *, *, #81163, .F. ) ;
#21813=DIRECTION ( 'NONE',  ( -4.274815082592931898E-19, -0.9999939076577903929, -0.003490651415223739937 ) ) ;
#21814=ADVANCED_FACE ( 'NONE', ( #8250 ), #128716, .T. ) ;
#21815=VERTEX_POINT ( 'NONE', #38389 ) ;
#21816=EDGE_LOOP ( 'NONE', ( #32836, #124643 ) ) ;
#21817=ORIENTED_EDGE ( 'NONE', *, *, #120813, .T. ) ;
#21818=AXIS2_PLACEMENT_3D ( 'NONE', #7859, #74679, #114590 ) ;
#21820=DIRECTION ( 'NONE',  ( 0.000000000000000000, -0.9999939076577903929, 0.003490651415223739937 ) ) ;
#21821=LINE ( 'NONE', #73470, #108585 ) ;
#21822=FACE_OUTER_BOUND ( 'NONE', #53129, .T. ) ;
#21823=CARTESIAN_POINT ( 'NONE',  ( 0.3999999999999568345, 2.500000000000000000, -4.922947341949753586 ) ) ;
#21824=ADVANCED_FACE ( 'NONE', ( #121426 ), #115759, .T. ) ;
#21825=FACE_OUTER_BOUND ( 'NONE', #122654, .T. ) ;
#21826=ADVANCED_FACE ( 'NONE', ( #81520 ), #82435, .T. ) ;
#21827=ADVANCED_FACE ( 'NONE', ( #61892 ), #90688, .T. ) ;
#21828=DIRECTION ( 'NONE',  ( -0.000000000000000000, 1.000000000000000000, -0.000000000000000000 ) ) ;
#21829=AXIS2_PLACEMENT_3D ( 'NONE', #114621, #34146, #105463 ) ;
#21830=CIRCLE ( 'NONE', #86653, 0.06509327318403745899 ) ;
#21831=EDGE_LOOP ( 'NONE', ( #101457, #42612 ) ) ;
#21832=DIRECTION ( 'NONE',  ( 0.000000000000000000, 0.000000000000000000, 1.000000000000000000 ) ) ;
#21833=ORIENTED_EDGE ( 'NONE', *, *, #21896, .T. ) ;
#21834=CARTESIAN_POINT ( 'NONE',  ( 4.799999999999935874, 2.500000000000000000, 0.3464101615137735735 ) ) ;
#21835=EDGE_CURVE ( 'NONE', #31016, #51588, #2960, .T. ) ;
#21836=VERTEX_POINT ( 'NONE', #50769 ) ;
#21837=CARTESIAN_POINT ( 'NONE',  ( -12.69999999999999396, 12.50000000000000000, -3.983716857408423628 ) ) ;
#21839=ORIENTED_EDGE ( 'NONE', *, *, #59248, .T. ) ;
#21840=ADVANCED_FACE ( 'NONE', ( #93271 ), #113720, .T. ) ;
#21841=DIRECTION ( 'NONE',  ( 0.000000000000000000, 0.000000000000000000, 1.000000000000000000 ) ) ;
#21842=EDGE_CURVE ( 'NONE', #45172, #21163, #31775, .T. ) ;
#21843=AXIS2_PLACEMENT_3D ( 'NONE', #108931, #109605, #30417 ) ;
#21844=ADVANCED_FACE ( 'NONE', ( #10803 ), #117909, .T. ) ;
#21845=DIRECTION ( 'NONE',  ( -4.274815082592931898E-19, -0.9999939076577903929, -0.003490651415223739937 ) ) ;
#21846=ORIENTED_EDGE ( 'NONE', *, *, #22729, .T. ) ;
#21847=ORIENTED_EDGE ( 'NONE', *, *, #54613, .F. ) ;
#21848=DIRECTION ( 'NONE',  ( 0.000000000000000000, 1.000000000000000000, 0.000000000000000000 ) ) ;
#21851=CARTESIAN_POINT ( 'NONE',  ( -3.950000000000025491, 2.500000000000000000, 6.148780366869520897 ) ) ;
#21852=ADVANCED_FACE ( 'NONE', ( #40970 ), #91977, .F. ) ;
#21853=CARTESIAN_POINT ( 'NONE',  ( -7.300000000000016698, 12.50000000000000000, -0.3464101615137783474 ) ) ;
#21854=ORIENTED_EDGE ( 'NONE', *, *, #63191, .T. ) ;
#21855=CIRCLE ( 'NONE', #5091, 0.06509327318403745899 ) ;
#21856=AXIS2_PLACEMENT_3D ( 'NONE', #5633, #106425, #45586 ) ;
#21857=DIRECTION ( 'NONE',  ( 0.000000000000000000, 0.000000000000000000, 1.000000000000000000 ) ) ;
#21858=B_SPLINE_CURVE_WITH_KNOTS ( 'NONE', 3,
 ( #26771, #128201, #66683, #38552, #87611, #106609, #85681, #126910, #125595, #66043, #105973, #109177, #111100, #51578, #61398, #69920 ),
 .UNSPECIFIED., .F., .F.,
 ( 4, 2, 2, 2, 2, 2, 2, 4 ),
 ( 0.0007527720032349511205, 0.001260609959331164412, 0.001768447915427377812, 0.002022366893475485271, 0.002276285871523592731, 0.002784123827619805047, 0.003799799739812229678, 0.004815475652004653877 ),
 .UNSPECIFIED. ) ;
#21859=CIRCLE ( 'NONE', #113786, 0.1000000000000000472 ) ;
#21860=ORIENTED_EDGE ( 'NONE', *, *, #80782, .F. ) ;
#21861=CIRCLE ( 'NONE', #115921, 0.06509327318403745899 ) ;
#21862=CARTESIAN_POINT ( 'NONE',  ( -11.25000000000000000, 12.50000000000000000, -2.857883832488649745 ) ) ;
#21863=LINE ( 'NONE', #91875, #81556 ) ;
#21865=DIRECTION ( 'NONE',  ( 0.000000000000000000, -0.000000000000000000, 1.000000000000000000 ) ) ;
#21866=DIRECTION ( 'NONE',  ( 0.000000000000000000, -0.9999939076577903929, 0.003490651415223739937 ) ) ;
#21867=CARTESIAN_POINT ( 'NONE',  ( -6.450000000000017941, 12.50000000000000000, -2.511473670974877948 ) ) ;
#21868=DIRECTION ( 'NONE',  ( 0.000000000000000000, 0.000000000000000000, 1.000000000000000000 ) ) ;
#21869=VERTEX_POINT ( 'NONE', #72983 ) ;
#21870=DIRECTION ( 'NONE',  ( 0.000000000000000000, -0.9999939076577903929, 0.003490651415223739937 ) ) ;
#21871=AXIS2_PLACEMENT_3D ( 'NONE', #72056, #9258, #100837 ) ;
#21872=DIRECTION ( 'NONE',  ( 0.000000000000000000, 0.000000000000000000, 1.000000000000000000 ) ) ;
#21873=CARTESIAN_POINT ( 'NONE',  ( -2.100000000000033396, 2.500000000000000000, -3.637306695894650055 ) ) ;
#21875=CONICAL_SURFACE ( 'NONE', #38509, 0.09999999999999982514, 0.003490658503988666988 ) ;
#21876=AXIS2_PLACEMENT_3D ( 'NONE', #16106, #113697, #44962 ) ;
#21877=EDGE_LOOP ( 'NONE', ( #64366, #105342, #115452, #105886 ) ) ;
#21878=DIRECTION ( 'NONE',  ( 0.000000000000000000, 1.000000000000000000, 0.000000000000000000 ) ) ;
#21879=CIRCLE ( 'NONE', #53180, 0.09999999999999982514 ) ;
#21880=ADVANCED_FACE ( 'NONE', ( #110950 ), #112909, .T. ) ;
#21881=EDGE_LOOP ( 'NONE', ( #83600, #89718, #59508, #126763 ) ) ;
#21882=AXIS2_PLACEMENT_3D ( 'NONE', #125949, #73626, #74933 ) ;
#21883=ORIENTED_EDGE ( 'NONE', *, *, #83616, .F. ) ;
#21884=DIRECTION ( 'NONE',  ( 0.000000000000000000, -0.9999939076577903929, 0.003490651415223739937 ) ) ;
#21885=CIRCLE ( 'NONE', #99246, 0.06509327318403745899 ) ;
#21886=ORIENTED_EDGE ( 'NONE', *, *, #62030, .T. ) ;
#21887=CARTESIAN_POINT ( 'NONE',  ( -2.300000000000032685, 12.50000000000000000, -0.4115034346978157509 ) ) ;
#21888=CARTESIAN_POINT ( 'NONE',  ( -8.750000000000005329, 2.500000000000000000, 5.802370205355744659 ) ) ;
#21889=CARTESIAN_POINT ( 'NONE',  ( 15.86953761860679712, 2.463355995079644867, 3.896699429477471721 ) ) ;
#21890=ORIENTED_EDGE ( 'NONE', *, *, #71847, .F. ) ;
#21891=VECTOR ( 'NONE', #94898, 1000.000000000000000 ) ;
#21892=AXIS2_PLACEMENT_3D ( 'NONE', #90303, #100767, #30781 ) ;
#21893=DIRECTION ( 'NONE',  ( 0.000000000000000000, 0.000000000000000000, -1.000000000000000000 ) ) ;
#21894=CARTESIAN_POINT ( 'NONE',  ( -1.900000000000034106, 12.50000000000000000, -4.048810130592463530 ) ) ;
#21895=AXIS2_PLACEMENT_3D ( 'NONE', #107133, #15528, #55477 ) ;
#21896=EDGE_CURVE ( 'NONE', #97929, #93847, #21294, .T. ) ;
#21897=EDGE_LOOP ( 'NONE', ( #16917, #109032, #124745, #58583 ) ) ;
#21898=EDGE_LOOP ( 'NONE', ( #32560, #44025 ) ) ;
#21899=ORIENTED_EDGE ( 'NONE', *, *, #26968, .T. ) ;
#21900=CARTESIAN_POINT ( 'NONE',  ( 0.3999999999999559464, 12.50000000000000000, -4.330127018922201643 ) ) ;
#21901=PLANE ( 'NONE',  #1929 ) ;
#21902=CARTESIAN_POINT ( 'NONE',  ( 5.849999999999933920, 12.50000000000000000, 5.802370205355744659 ) ) ;
#21903=FACE_BOUND ( 'NONE', #24417, .T. ) ;
#21904=ORIENTED_EDGE ( 'NONE', *, *, #15276, .T. ) ;
#21905=CARTESIAN_POINT ( 'NONE',  ( -6.250000000000021316, 2.500000000000000000, -5.902370205355750521 ) ) ;
#21907=VECTOR ( 'NONE', #110985, 1000.000000000000000 ) ;
#21908=VERTEX_POINT ( 'NONE', #120789 ) ;
#21909=CARTESIAN_POINT ( 'NONE',  ( 8.949999999999917577, 12.50000000000000000, -2.511473670974877948 ) ) ;
#21910=DIRECTION ( 'NONE',  ( -0.000000000000000000, -1.000000000000000000, -0.000000000000000000 ) ) ;
#21911=LINE ( 'NONE', #12068, #115462 ) ;
#21912=DIRECTION ( 'NONE',  ( -0.000000000000000000, -1.000000000000000000, -0.000000000000000000 ) ) ;
#21913=CARTESIAN_POINT ( 'NONE',  ( -8.750000000000010658, 2.500000000000000000, -7.088010851410848190 ) ) ;
#21914=DIRECTION ( 'NONE',  ( 0.000000000000000000, 0.000000000000000000, 1.000000000000000000 ) ) ;
#21915=DIRECTION ( 'NONE',  ( 0.000000000000000000, 0.000000000000000000, 1.000000000000000000 ) ) ;
#21916=CIRCLE ( 'NONE', #97118, 0.06509327318403741736 ) ;
#21917=EDGE_CURVE ( 'NONE', #108081, #18231, #846, .T. ) ;
#21918=ORIENTED_EDGE ( 'NONE', *, *, #4313, .F. ) ;
#21919=EDGE_LOOP ( 'NONE', ( #34325, #57345 ) ) ;
#21920=ORIENTED_EDGE ( 'NONE', *, *, #76289, .T. ) ;
#21921=ORIENTED_EDGE ( 'NONE', *, *, #127946, .F. ) ;
#21922=PLANE ( 'NONE',  #128973 ) ;
#21923=DIRECTION ( 'NONE',  ( -0.000000000000000000, 1.000000000000000000, -0.000000000000000000 ) ) ;
#21924=ORIENTED_EDGE ( 'NONE', *, *, #77270, .T. ) ;
#21925=FACE_BOUND ( 'NONE', #124769, .T. ) ;
#21926=ADVANCED_FACE ( 'NONE', ( #32443 ), #23225, .T. ) ;
#21927=CARTESIAN_POINT ( 'NONE',  ( -13.09999999999999254, 12.50000000000000000, 0.4115034346978151958 ) ) ;
#21928=DIRECTION ( 'NONE',  ( -0.000000000000000000, 1.000000000000000000, -0.000000000000000000 ) ) ;
#21929=CIRCLE ( 'NONE', #80419, 0.09999999999999999167 ) ;
#21930=DIRECTION ( 'NONE',  ( 0.000000000000000000, 0.000000000000000000, 1.000000000000000000 ) ) ;
#21931=CARTESIAN_POINT ( 'NONE',  ( -9.600000000000008527, 12.50000000000000000, -5.088040615133786915 ) ) ;
#21932=VECTOR ( 'NONE', #7230, 1000.000000000000000 ) ;
#21933=DIRECTION ( 'NONE',  ( -0.000000000000000000, 1.000000000000000000, -0.000000000000000000 ) ) ;
#21934=EDGE_CURVE ( 'NONE', #702, #78294, #101160, .T. ) ;
#21935=DIRECTION ( 'NONE',  ( -0.000000000000000000, -1.000000000000000000, -0.000000000000000000 ) ) ;
#21936=EDGE_CURVE ( 'NONE', #72308, #48106, #91332, .T. ) ;
#21937=LINE ( 'NONE', #62509, #39187 ) ;
#21938=CARTESIAN_POINT ( 'NONE',  ( 13.94999999999989271, 2.500000000000000000, -1.918653347947326004 ) ) ;
#21939=EDGE_CURVE ( 'NONE', #106700, #100735, #94939, .T. ) ;
#21940=DIRECTION ( 'NONE',  ( -0.000000000000000000, -1.000000000000000000, -0.000000000000000000 ) ) ;
#21941=EDGE_CURVE ( 'NONE', #67379, #46379, #25885, .T. ) ;
#21942=ORIENTED_EDGE ( 'NONE', *, *, #79466, .T. ) ;
#21943=EDGE_CURVE ( 'NONE', #112402, #111058, #87780, .T. ) ;
#21944=VERTEX_POINT ( 'NONE', #27566 ) ;
#21945=AXIS2_PLACEMENT_3D ( 'NONE', #20275, #110585, #14768 ) ;
#21946=ORIENTED_EDGE ( 'NONE', *, *, #110607, .T. ) ;
#21947=VERTEX_POINT ( 'NONE', #35642 ) ;
#21948=VECTOR ( 'NONE', #98519, 1000.000000000000000 ) ;
#21949=ORIENTED_EDGE ( 'NONE', *, *, #101012, .F. ) ;
#21950=ORIENTED_EDGE ( 'NONE', *, *, #83749, .T. ) ;
#21951=ORIENTED_EDGE ( 'NONE', *, *, #46811, .F. ) ;
#21952=CARTESIAN_POINT ( 'NONE',  ( 9.799999999999913669, 12.50000000000000000, 4.611443907251934426 ) ) ;
#21953=VECTOR ( 'NONE', #4343, 1000.000000000000000 ) ;
#21954=ORIENTED_EDGE ( 'NONE', *, *, #46216, .F. ) ;
#21955=EDGE_CURVE ( 'NONE', #37658, #87328, #90735, .T. ) ;
#21956=VERTEX_POINT ( 'NONE', #53989 ) ;
#21957=CIRCLE ( 'NONE', #5190, 0.06509327318403745899 ) ;
#21958=ADVANCED_FACE ( 'NONE', ( #14041 ), #76066, .T. ) ;
#21959=ADVANCED_FACE ( 'NONE', ( #14681 ), #19630, .T. ) ;
#21960=DIRECTION ( 'NONE',  ( -0.000000000000000000, 1.000000000000000000, -0.000000000000000000 ) ) ;
#21961=CARTESIAN_POINT ( 'NONE',  ( 14.93723468939153420, -2.500000000000000444, 6.174425106950333308 ) ) ;
#21962=DIRECTION ( 'NONE',  ( -0.000000000000000000, 1.000000000000000000, -0.000000000000000000 ) ) ;
#21963=CARTESIAN_POINT ( 'NONE',  ( 9.149999999999918643, 2.500000000000000000, -6.595190528383302109 ) ) ;
#21964=ORIENTED_EDGE ( 'NONE', *, *, #61010, .T. ) ;
#21965=DIRECTION ( 'NONE',  ( -0.000000000000000000, -1.000000000000000000, -0.000000000000000000 ) ) ;
#21966=VERTEX_POINT ( 'NONE', #93916 ) ;
#21967=CONICAL_SURFACE ( 'NONE', #72124, 0.09999999999999982514, 0.003490658503988666988 ) ;
#21968=ORIENTED_EDGE ( 'NONE', *, *, #106467, .F. ) ;
#21969=DIRECTION ( 'NONE',  ( 0.000000000000000000, -0.9999939076577903929, 0.003490651415223739937 ) ) ;
#21970=CIRCLE ( 'NONE', #7259, 0.06509327318403745899 ) ;
#21972=DIRECTION ( 'NONE',  ( 0.000000000000000000, 0.000000000000000000, 1.000000000000000000 ) ) ;
#21973=ORIENTED_EDGE ( 'NONE', *, *, #98410, .F. ) ;
#21974=EDGE_LOOP ( 'NONE', ( #72200, #97243, #128332, #42716 ) ) ;
#21975=CARTESIAN_POINT ( 'NONE',  ( -8.350000000000013856, 12.50000000000000000, -7.122917578226811486 ) ) ;
#21976=AXIS2_PLACEMENT_3D ( 'NONE', #105184, #44995, #26632 ) ;
#21977=CONICAL_SURFACE ( 'NONE', #105585, 0.1000000000000002554, 0.003490658503988666988 ) ;
#21978=VECTOR ( 'NONE', #77503, 1000.000000000000000 ) ;
#21979=DIRECTION ( 'NONE',  ( 0.000000000000000000, -0.000000000000000000, 1.000000000000000000 ) ) ;
#21980=DIRECTION ( 'NONE',  ( 0.000000000000000000, 1.000000000000000000, 0.000000000000000000 ) ) ;
#21981=CARTESIAN_POINT ( 'NONE',  ( 3.749999999999944045, 2.500000000000000000, -7.288010851410854585 ) ) ;
#21982=ADVANCED_FACE ( 'NONE', ( #67482 ), #88673, .T. ) ;
#21983=CIRCLE ( 'NONE', #74192, 0.06509327318403745899 ) ;
#21984=DIRECTION ( 'NONE',  ( 0.000000000000000000, 0.000000000000000000, 1.000000000000000000 ) ) ;
#21985=EDGE_LOOP ( 'NONE', ( #44848, #33587, #24089, #125288 ) ) ;
#21986=DIRECTION ( 'NONE',  ( 0.000000000000000000, 0.000000000000000000, -1.000000000000000000 ) ) ;
#21987=AXIS2_PLACEMENT_3D ( 'NONE', #75107, #74462, #3787 ) ;
#21988=CIRCLE ( 'NONE', #82614, 0.06509327318403745899 ) ;
#21989=ORIENTED_EDGE ( 'NONE', *, *, #110150, .T. ) ;
#21990=DIRECTION ( 'NONE',  ( -0.000000000000000000, -1.000000000000000000, -0.000000000000000000 ) ) ;
#21991=DIRECTION ( 'NONE',  ( 0.000000000000000000, 1.000000000000000000, 0.000000000000000000 ) ) ;
#21992=FACE_OUTER_BOUND ( 'NONE', #3260, .T. ) ;
#21993=CIRCLE ( 'NONE', #11506, 0.06509327318403745899 ) ;
#21994=CARTESIAN_POINT ( 'NONE',  ( -7.499999999999976907, 12.50000000000000000, 4.330127018922196314 ) ) ;
#21995=EDGE_CURVE ( 'NONE', #128788, #22282, #11307, .T. ) ;
#21996=CARTESIAN_POINT ( 'NONE',  ( -15.59999999999998010, 2.500000000000000000, -0.3464101615137759604 ) ) ;
#21997=VERTEX_POINT ( 'NONE', #55280 ) ;
#21998=EDGE_CURVE ( 'NONE', #17511, #101710, #107436, .T. ) ;
#21999=CARTESIAN_POINT ( 'NONE',  ( 9.799999999999918998, 2.500000000000000000, -0.2464101615137782308 ) ) ;
#22000=EDGE_CURVE ( 'NONE', #106597, #7810, #111670, .T. ) ;
#22001=LINE ( 'NONE', #90716, #113438 ) ;
#22002=ORIENTED_EDGE ( 'NONE', *, *, #105094, .F. ) ;
#22003=ORIENTED_EDGE ( 'NONE', *, *, #63743, .F. ) ;
#22004=EDGE_LOOP ( 'NONE', ( #53366, #14114, #110571, #14884 ) ) ;
#22005=DIRECTION ( 'NONE',  ( 0.000000000000000000, 1.000000000000000000, 0.000000000000000000 ) ) ;
#22006=FACE_OUTER_BOUND ( 'NONE', #102096, .T. ) ;
#22008=CIRCLE ( 'NONE', #63756, 0.09999999999999982514 ) ;
#22009=CARTESIAN_POINT ( 'NONE',  ( 3.949999999999938893, 2.500000000000000000, 6.248780366869520542 ) ) ;
#22010=EDGE_CURVE ( 'NONE', #42781, #125134, #74920, .T. ) ;
#22011=DIRECTION ( 'NONE',  ( 0.000000000000000000, 0.000000000000000000, 1.000000000000000000 ) ) ;
#22012=CARTESIAN_POINT ( 'NONE',  ( -13.09999999999999254, 12.50000000000000000, -0.3464101615137741286 ) ) ;
#22013=DIRECTION ( 'NONE',  ( 0.000000000000000000, -0.9999939076577903929, 0.003490651415223739937 ) ) ;
#22014=CARTESIAN_POINT ( 'NONE',  ( -2.050000000000032685, 2.500000000000000000, -6.495190528383302464 ) ) ;
#22015=AXIS2_PLACEMENT_3D ( 'NONE', #92427, #2753, #40116 ) ;
#22016=CIRCLE ( 'NONE', #128546, 0.06509327318403745899 ) ;
#22017=ORIENTED_EDGE ( 'NONE', *, *, #2145, .T. ) ;
#22018=DIRECTION ( 'NONE',  ( 0.000000000000000000, 0.000000000000000000, -1.000000000000000000 ) ) ;
#22019=CARTESIAN_POINT ( 'NONE',  ( 2.699999999999947331, 2.500000000000000000, -4.676537180435978769 ) ) ;
#22020=EDGE_CURVE ( 'NONE', #55645, #12624, #105401, .T. ) ;
#22021=CARTESIAN_POINT ( 'NONE',  ( 4.999999999999933387, 2.500000000000000000, 5.022947341949748790 ) ) ;
#22022=CARTESIAN_POINT ( 'NONE',  ( 0.5999999999999555689, 2.500000000000000000, 4.676537180435972552 ) ) ;
#22023=ORIENTED_EDGE ( 'NONE', *, *, #97778, .F. ) ;
#22024=DIRECTION ( 'NONE',  ( -4.274815082592931898E-19, -0.9999939076577903929, -0.003490651415223739937 ) ) ;
#22025=AXIS2_PLACEMENT_3D ( 'NONE', #127636, #16366, #66771 ) ;
#22026=AXIS2_PLACEMENT_3D ( 'NONE', #64723, #56188, #123633 ) ;
#22027=CARTESIAN_POINT ( 'NONE',  ( -10.45000000000000107, 2.500000000000000000, 2.265063509461097357 ) ) ;
#22028=CARTESIAN_POINT ( 'NONE',  ( 0.000000000000000000, 2.500000000000000000, 0.000000000000000000 ) ) ;
#22029=ORIENTED_EDGE ( 'NONE', *, *, #98310, .F. ) ;
#22030=ORIENTED_EDGE ( 'NONE', *, *, #69193, .T. ) ;
#22031=FACE_OUTER_BOUND ( 'NONE', #84302, .T. ) ;
#22032=CONICAL_SURFACE ( 'NONE', #3243, 0.09999999999999982514, 0.003490658503988666988 ) ;
#22033=AXIS2_PLACEMENT_3D ( 'NONE', #6750, #84046, #15293 ) ;
#22034=ADVANCED_FACE ( 'NONE', ( #47887 ), #124009, .T. ) ;
#22035=EDGE_LOOP ( 'NONE', ( #112711, #105125, #24153, #53753 ) ) ;
#22036=VERTEX_POINT ( 'NONE', #127716 ) ;
#22037=CARTESIAN_POINT ( 'NONE',  ( 11.44999999999990692, 2.500000000000000000, -6.841600689897078702 ) ) ;
#22038=EDGE_CURVE ( 'NONE', #125864, #88124, #38057, .T. ) ;
#22039=DIRECTION ( 'NONE',  ( 0.000000000000000000, 1.000000000000000000, 0.000000000000000000 ) ) ;
#22040=DIRECTION ( 'NONE',  ( 0.000000000000000000, 0.000000000000000000, -1.000000000000000000 ) ) ;
#22041=LINE ( 'NONE', #121490, #62562 ) ;
#22042=ORIENTED_EDGE ( 'NONE', *, *, #28444, .T. ) ;
#22043=CIRCLE ( 'NONE', #111913, 0.1000000000000002554 ) ;
#22044=CARTESIAN_POINT ( 'NONE',  ( -4.350000000000023626, 12.50000000000000000, 1.818653347947321475 ) ) ;
#22046=CARTESIAN_POINT ( 'NONE',  ( 17.50000000000011013, 2.262036863575971335, 3.993716676843428015 ) ) ;
#22047=EDGE_CURVE ( 'NONE', #29184, #121009, #23837, .T. ) ;
#22048=CARTESIAN_POINT ( 'NONE',  ( -6.250000000000019540, 2.500000000000000000, -2.957883832488653830 ) ) ;
#22049=CIRCLE ( 'NONE', #99311, 0.1000000000000002554 ) ;
#22050=ORIENTED_EDGE ( 'NONE', *, *, #72344, .T. ) ;
#22051=CIRCLE ( 'NONE', #57551, 0.06509327318403745899 ) ;
#22052=ORIENTED_EDGE ( 'NONE', *, *, #119170, .T. ) ;
#22054=ORIENTED_EDGE ( 'NONE', *, *, #36591, .F. ) ;
#22055=EDGE_LOOP ( 'NONE', ( #21756, #59529, #23883, #78552 ) ) ;
#22056=CARTESIAN_POINT ( 'NONE',  ( -9.600000000000008527, 12.50000000000000000, -0.06509327318403980434 ) ) ;
#22057=CARTESIAN_POINT ( 'NONE',  ( 15.40585131749456949, 2.500000000000000000, 5.817868756320654811 ) ) ;
#22058=DIRECTION ( 'NONE',  ( 0.000000000000000000, 0.000000000000000000, 1.000000000000000000 ) ) ;
#22059=FACE_BOUND ( 'NONE', #63542, .T. ) ;
#22060=ORIENTED_EDGE ( 'NONE', *, *, #50028, .F. ) ;
#22061=DIRECTION ( 'NONE',  ( 0.000000000000000000, -0.000000000000000000, 1.000000000000000000 ) ) ;
#22063=CARTESIAN_POINT ( 'NONE',  ( -11.84999999999999787, 12.50000000000000000, -1.818653347947321919 ) ) ;
#22064=CARTESIAN_POINT ( 'NONE',  ( 12.49999999999993605, 2.500000000000000000, -2.276824562219559311E-15 ) ) ;
#22065=AXIS2_PLACEMENT_3D ( 'NONE', #74138, #4090, #23098 ) ;
#22066=AXIS2_PLACEMENT_3D ( 'NONE', #17568, #108541, #50273 ) ;
#22067=CONICAL_SURFACE ( 'NONE', #19915, 0.1000000000000000472, 0.003490658503988666988 ) ;
#22068=CARTESIAN_POINT ( 'NONE',  ( -12.49999999999999289, 2.500000000000000000, 4.922947341949748257 ) ) ;
#22069=CONICAL_SURFACE ( 'NONE', #7365, 0.1000000000000000472, 0.003490658503988666988 ) ;
#22070=DIRECTION ( 'NONE',  ( -0.000000000000000000, -1.000000000000000000, -0.000000000000000000 ) ) ;
#22071=FACE_OUTER_BOUND ( 'NONE', #1001, .T. ) ;
#22072=CIRCLE ( 'NONE', #76437, 0.06509327318403745899 ) ;
#22073=DIRECTION ( 'NONE',  ( -0.000000000000000000, 1.000000000000000000, -0.000000000000000000 ) ) ;
#22074=AXIS2_PLACEMENT_3D ( 'NONE', #76849, #127869, #97768 ) ;
#22075=ADVANCED_FACE ( 'NONE', ( #58356 ), #59159, .T. ) ;
#22076=ORIENTED_EDGE ( 'NONE', *, *, #30499, .F. ) ;
#22077=ORIENTED_EDGE ( 'NONE', *, *, #50450, .T. ) ;
#22078=EDGE_LOOP ( 'NONE', ( #69342, #29103 ) ) ;
#22079=EDGE_LOOP ( 'NONE', ( #52472, #35518, #97164, #109649 ) ) ;
#22081=DIRECTION ( 'NONE',  ( -0.000000000000000000, 1.000000000000000000, -0.000000000000000000 ) ) ;
#22082=PLANE ( 'NONE',  #17327 ) ;
#22083=ORIENTED_EDGE ( 'NONE', *, *, #48287, .F. ) ;
#22084=FACE_BOUND ( 'NONE', #93430, .T. ) ;
#22085=DIRECTION ( 'NONE',  ( -0.000000000000000000, -1.000000000000000000, -0.000000000000000000 ) ) ;
#22086=ADVANCED_FACE ( 'NONE', ( #28240 ), #68145, .T. ) ;
#22087=ORIENTED_EDGE ( 'NONE', *, *, #16900, .T. ) ;
#22088=EDGE_CURVE ( 'NONE', #77067, #51687, #113548, .T. ) ;
#22089=DIRECTION ( 'NONE',  ( -4.274815082592931898E-19, -0.9999939076577903929, -0.003490651415223739937 ) ) ;
#22090=ADVANCED_FACE ( 'NONE', ( #30185 ), #103049, .T. ) ;
#22091=DIRECTION ( 'NONE',  ( -0.000000000000000000, -1.000000000000000000, -0.000000000000000000 ) ) ;
#22092=EDGE_CURVE ( 'NONE', #110447, #89399, #23629, .T. ) ;
#22093=DIRECTION ( 'NONE',  ( 0.000000000000000000, 0.000000000000000000, 1.000000000000000000 ) ) ;
#22094=EDGE_CURVE ( 'NONE', #72573, #36539, #75852, .T. ) ;
#22095=CIRCLE ( 'NONE', #95245, 0.06509327318403745899 ) ;
#22096=VERTEX_POINT ( 'NONE', #31465 ) ;
#22097=DIRECTION ( 'NONE',  ( -0.000000000000000000, 1.000000000000000000, -0.000000000000000000 ) ) ;
#22098=ORIENTED_EDGE ( 'NONE', *, *, #47377, .F. ) ;
#22099=VERTEX_POINT ( 'NONE', #1342 ) ;
#22100=ADVANCED_FACE ( 'NONE', ( #21640 ), #27828, .T. ) ;
#22101=ORIENTED_EDGE ( 'NONE', *, *, #96858, .T. ) ;
#22102=FACE_OUTER_BOUND ( 'NONE', #72278, .T. ) ;
#22103=ADVANCED_FACE ( 'NONE', ( #99566 ), #115549, .T. ) ;
#22104=DIRECTION ( 'NONE',  ( 0.000000000000000000, 0.000000000000000000, 1.000000000000000000 ) ) ;
#22105=CIRCLE ( 'NONE', #97300, 0.1000000000000002554 ) ;
#22106=ORIENTED_EDGE ( 'NONE', *, *, #18236, .F. ) ;
#22107=ADVANCED_FACE ( 'NONE', ( #11159 ), #6876, .T. ) ;
#22108=DIRECTION ( 'NONE',  ( -4.274815082592931898E-19, -0.9999939076577903929, -0.003490651415223739937 ) ) ;
#22109=AXIS2_PLACEMENT_3D ( 'NONE', #129174, #28375, #79413 ) ;
#22110=AXIS2_PLACEMENT_3D ( 'NONE', #25250, #65173, #64547 ) ;
#22111=ADVANCED_FACE ( 'NONE', ( #108719 ), #11093, .T. ) ;
#22112=CARTESIAN_POINT ( 'NONE',  ( 10.64999999999991331, 2.500000000000000000, -2.511473670974877948 ) ) ;
#22113=EDGE_CURVE ( 'NONE', #103547, #30982, #119833, .T. ) ;
#22114=DIRECTION ( 'NONE',  ( 0.000000000000000000, 0.000000000000000000, 1.000000000000000000 ) ) ;
#22115=CARTESIAN_POINT ( 'NONE',  ( 10.44999999999991402, 12.50000000000000000, 6.495190528383297135 ) ) ;
#22117=ORIENTED_EDGE ( 'NONE', *, *, #2864, .F. ) ;
#22118=CARTESIAN_POINT ( 'NONE',  ( -7.500000000000001776, 1.500000000000000000, 1.734723475976807094E-15 ) ) ;
#22119=EDGE_CURVE ( 'NONE', #41869, #7747, #49827, .T. ) ;
#22120=ORIENTED_EDGE ( 'NONE', *, *, #114538, .F. ) ;
#22121=CARTESIAN_POINT ( 'NONE',  ( 11.44999999999991047, 2.500000000000000000, 6.148780366869520009 ) ) ;
#22122=VECTOR ( 'NONE', #76608, 1000.000000000000000 ) ;
#22123=ORIENTED_EDGE ( 'NONE', *, *, #48529, .T. ) ;
#22124=CIRCLE ( 'NONE', #19954, 0.06509327318403745899 ) ;
#22125=DIRECTION ( 'NONE',  ( -0.000000000000000000, 1.000000000000000000, -0.000000000000000000 ) ) ;
#22126=ORIENTED_EDGE ( 'NONE', *, *, #46022, .T. ) ;
#22127=DIRECTION ( 'NONE',  ( 0.000000000000000000, 0.000000000000000000, 1.000000000000000000 ) ) ;
#22128=DIRECTION ( 'NONE',  ( -0.000000000000000000, -1.000000000000000000, -0.000000000000000000 ) ) ;
#22129=DIRECTION ( 'NONE',  ( 0.000000000000000000, -0.000000000000000000, 1.000000000000000000 ) ) ;
#22130=DIRECTION ( 'NONE',  ( 0.000000000000000000, 0.000000000000000000, 1.000000000000000000 ) ) ;
#22131=PLANE ( 'NONE',  #24459 ) ;
#22132=ORIENTED_EDGE ( 'NONE', *, *, #79002, .T. ) ;
#22133=EDGE_LOOP ( 'NONE', ( #41049, #129067 ) ) ;
#22134=DIRECTION ( 'NONE',  ( 0.000000000000000000, -0.000000000000000000, 1.000000000000000000 ) ) ;
#22135=CIRCLE ( 'NONE', #107791, 0.06509327318403745899 ) ;
#22136=VECTOR ( 'NONE', #104188, 1000.000000000000000 ) ;
#22137=CARTESIAN_POINT ( 'NONE',  ( 9.399999999999918643, 2.500000000000000000, 0.4464101615137736623 ) ) ;
#22138=DIRECTION ( 'NONE',  ( 0.000000000000000000, 0.000000000000000000, 1.000000000000000000 ) ) ;
#22139=EDGE_LOOP ( 'NONE', ( #57115, #111686 ) ) ;
#22140=VERTEX_POINT ( 'NONE', #110655 ) ;
#22141=ORIENTED_EDGE ( 'NONE', *, *, #65149, .T. ) ;
#22142=CARTESIAN_POINT ( 'NONE',  ( 3.149999999999942624, 12.50000000000000000, 6.841600689897072485 ) ) ;
#22143=EDGE_LOOP ( 'NONE', ( #60107, #33101, #66086, #84375 ) ) ;
#22144=DIRECTION ( 'NONE',  ( 0.000000000000000000, 0.000000000000000000, 1.000000000000000000 ) ) ;
#22145=DIRECTION ( 'NONE',  ( -0.000000000000000000, -1.000000000000000000, -0.000000000000000000 ) ) ;
#22146=LINE ( 'NONE', #41787, #86603 ) ;
#22147=ORIENTED_EDGE ( 'NONE', *, *, #41477, .F. ) ;
#22148=CARTESIAN_POINT ( 'NONE',  ( -11.05000000000000071, 12.50000000000000000, 6.841600689897072485 ) ) ;
#22149=DIRECTION ( 'NONE',  ( 0.000000000000000000, 0.000000000000000000, 1.000000000000000000 ) ) ;
#22150=CARTESIAN_POINT ( 'NONE',  ( -6.650000000000015454, 2.500000000000000000, 2.857883832488649301 ) ) ;
#22151=FACE_OUTER_BOUND ( 'NONE', #9147, .T. ) ;
#22152=DIRECTION ( 'NONE',  ( -0.000000000000000000, 1.000000000000000000, -0.000000000000000000 ) ) ;
#22153=ORIENTED_EDGE ( 'NONE', *, *, #62853, .T. ) ;
#22154=ADVANCED_FACE ( 'NONE', ( #111279 ), #19414, .T. ) ;
#22155=CARTESIAN_POINT ( 'NONE',  ( 4.199999999999941558, 2.500000000000000000, -4.430127018922202176 ) ) ;
#22156=AXIS2_PLACEMENT_3D ( 'NONE', #23062, #92438, #91801 ) ;
#22157=VECTOR ( 'NONE', #90565, 1000.000000000000000 ) ;
#22158=FACE_OUTER_BOUND ( 'NONE', #81583, .T. ) ;
#22159=ADVANCED_FACE ( 'NONE', ( #79911 ), #81211, .T. ) ;
#22160=EDGE_LOOP ( 'NONE', ( #83291, #83022, #84538, #101307 ) ) ;
#22161=VERTEX_POINT ( 'NONE', #89093 ) ;
#22163=DIRECTION ( 'NONE',  ( 0.000000000000000000, -0.9999939076577903929, 0.003490651415223739937 ) ) ;
#22164=CARTESIAN_POINT ( 'NONE',  ( 6.699999999999928235, 2.500000000000000000, -2.276824562219559311E-15 ) ) ;
#22165=FACE_OUTER_BOUND ( 'NONE', #124957, .T. ) ;
#22166=ADVANCED_FACE ( 'NONE', ( #118535 ), #73800, .T. ) ;
#22167=CARTESIAN_POINT ( 'NONE',  ( -10.65000000000000213, 2.500000000000000000, 2.511473670974873507 ) ) ;
#22168=EDGE_CURVE ( 'NONE', #118189, #39604, #100822, .T. ) ;
#22169=DIRECTION ( 'NONE',  ( 0.000000000000000000, 0.000000000000000000, 1.000000000000000000 ) ) ;
#22170=CARTESIAN_POINT ( 'NONE',  ( 1.899999999999951283, 12.50000000000000000, -0.2813168883297408329 ) ) ;
#22171=LINE ( 'NONE', #42444, #120906 ) ;
#22172=CIRCLE ( 'NONE', #9619, 0.06509327318403745899 ) ;
#22173=CARTESIAN_POINT ( 'NONE',  ( -0.8500000000000390576, 2.500000000000000000, -2.165063509461101710 ) ) ;
#22174=AXIS2_PLACEMENT_3D ( 'NONE', #101685, #121316, #19232 ) ;
#22175=AXIS2_PLACEMENT_3D ( 'NONE', #1948, #22271, #91630 ) ;
#22176=EDGE_LOOP ( 'NONE', ( #74624, #16150 ) ) ;
#22177=ORIENTED_EDGE ( 'NONE', *, *, #44319, .F. ) ;
#22178=ORIENTED_EDGE ( 'NONE', *, *, #50281, .F. ) ;
#22179=CONICAL_SURFACE ( 'NONE', #95315, 0.1000000000000002554, 0.003490658503988666988 ) ;
#22180=VERTEX_POINT ( 'NONE', #29529 ) ;
#22181=CARTESIAN_POINT ( 'NONE',  ( 5.199999999999937117, 2.500000000000000000, -4.776537180435978414 ) ) ;
#22182=LINE ( 'NONE', #102639, #123136 ) ;
#22183=EDGE_LOOP ( 'NONE', ( #51900, #121292 ) ) ;
#22184=DIRECTION ( 'NONE',  ( -0.000000000000000000, -1.000000000000000000, -0.000000000000000000 ) ) ;
#22185=PLANE ( 'NONE',  #101574 ) ;
#22186=CARTESIAN_POINT ( 'NONE',  ( 5.849999999999935696, 2.500000000000000000, -6.395190528383301931 ) ) ;
#22187=VERTEX_POINT ( 'NONE', #51113 ) ;
#22188=FACE_OUTER_BOUND ( 'NONE', #28766, .T. ) ;
#22189=CIRCLE ( 'NONE', #122518, 0.06509327318403745899 ) ;
#22190=FACE_OUTER_BOUND ( 'NONE', #111692, .T. ) ;
#22191=ADVANCED_FACE ( 'NONE', ( #39371 ), #36173, .T. ) ;
#22192=EDGE_LOOP ( 'NONE', ( #35377, #96186, #95894, #3351 ) ) ;
#22193=ORIENTED_EDGE ( 'NONE', *, *, #46305, .F. ) ;
#22194=ORIENTED_EDGE ( 'NONE', *, *, #4265, .F. ) ;
#22195=ORIENTED_EDGE ( 'NONE', *, *, #97283, .F. ) ;
#22196=CARTESIAN_POINT ( 'NONE',  ( 1.849999999999949685, 2.500000000000000000, -2.511473670974877948 ) ) ;
#22197=CIRCLE ( 'NONE', #38934, 0.06509327318403743123 ) ;
#22198=AXIS2_PLACEMENT_3D ( 'NONE', #19817, #70200, #87881 ) ;
#22199=CARTESIAN_POINT ( 'NONE',  ( 6.649999999999931966, 2.500000000000000000, -7.288010851410854585 ) ) ;
#22200=CARTESIAN_POINT ( 'NONE',  ( 10.84999999999990905, 2.500000000000000000, 1.372243186433545370 ) ) ;
#22201=EDGE_LOOP ( 'NONE', ( #46484, #112101 ) ) ;
#22202=CIRCLE ( 'NONE', #95344, 0.1000000000000002554 ) ;
#22203=DIRECTION ( 'NONE',  ( 0.000000000000000000, 0.000000000000000000, 1.000000000000000000 ) ) ;
#22204=EDGE_CURVE ( 'NONE', #124884, #20780, #59664, .T. ) ;
#22205=VERTEX_POINT ( 'NONE', #38732 ) ;
#22206=DIRECTION ( 'NONE',  ( 0.000000000000000000, 1.000000000000000000, 0.000000000000000000 ) ) ;
#22207=CARTESIAN_POINT ( 'NONE',  ( 3.677919667776838875, -2.499999999999999556, -8.999999999883526058 ) ) ;
#22208=DIRECTION ( 'NONE',  ( -0.000000000000000000, -1.000000000000000000, -0.000000000000000000 ) ) ;
#22209=DIRECTION ( 'NONE',  ( 0.000000000000000000, 0.000000000000000000, -1.000000000000000000 ) ) ;
#22210=ADVANCED_FACE ( 'NONE', ( #78644 ), #119775, .T. ) ;
#22211=AXIS2_PLACEMENT_3D ( 'NONE', #107845, #117638, #38488 ) ;
#22212=VERTEX_POINT ( 'NONE', #13733 ) ;
#22213=AXIS2_PLACEMENT_3D ( 'NONE', #10497, #100188, #91008 ) ;
#22214=AXIS2_PLACEMENT_3D ( 'NONE', #121894, #34171, #114017 ) ;
#22215=ORIENTED_EDGE ( 'NONE', *, *, #109575, .T. ) ;
#22216=VERTEX_POINT ( 'NONE', #121760 ) ;
#22217=DIRECTION ( 'NONE',  ( 0.000000000000000000, 0.000000000000000000, -1.000000000000000000 ) ) ;
#22218=FACE_OUTER_BOUND ( 'NONE', #82196, .T. ) ;
#22219=EDGE_CURVE ( 'NONE', #7581, #39960, #44565, .T. ) ;
#22220=CARTESIAN_POINT ( 'NONE',  ( 1.849999999999948130, 2.500000000000000000, 6.148780366869520009 ) ) ;
#22221=FACE_BOUND ( 'NONE', #82615, .T. ) ;
#22222=CARTESIAN_POINT ( 'NONE',  ( 7.899999999999923084, 2.500000000000000000, -0.5928203230275542746 ) ) ;
#22223=DIRECTION ( 'NONE',  ( 0.000000000000000000, 1.000000000000000000, 0.000000000000000000 ) ) ;
#22224=CARTESIAN_POINT ( 'NONE',  ( -2.700000000000029932, 2.500000000000000000, -0.2464101615137782308 ) ) ;
#22225=DIRECTION ( 'NONE',  ( 0.000000000000000000, -0.9999939076577903929, 0.003490651415223739937 ) ) ;
#22226=FACE_OUTER_BOUND ( 'NONE', #71483, .T. ) ;
#22227=DIRECTION ( 'NONE',  ( 0.000000000000000000, -0.000000000000000000, 1.000000000000000000 ) ) ;
#22228=EDGE_LOOP ( 'NONE', ( #6153, #42495, #101289, #89419 ) ) ;
#22229=FACE_OUTER_BOUND ( 'NONE', #45379, .T. ) ;
#22230=DIRECTION ( 'NONE',  ( 0.000000000000000000, 0.000000000000000000, 1.000000000000000000 ) ) ;
#22231=VERTEX_POINT ( 'NONE', #34703 ) ;
#22232=ORIENTED_EDGE ( 'NONE', *, *, #66381, .F. ) ;
#22233=FACE_OUTER_BOUND ( 'NONE', #76771, .T. ) ;
#22234=FACE_OUTER_BOUND ( 'NONE', #118501, .T. ) ;
#22235=FACE_BOUND ( 'NONE', #92804, .T. ) ;
#22236=DIRECTION ( 'NONE',  ( -4.274815082592931898E-19, -0.9999939076577903929, -0.003490651415223739937 ) ) ;
#22237=ADVANCED_FACE ( 'NONE', ( #92300 ), #111344, .T. ) ;
#22238=VECTOR ( 'NONE', #85829, 1000.000000000000000 ) ;
#22239=AXIS2_PLACEMENT_3D ( 'NONE', #56280, #44536, #64172 ) ;
#22240=ORIENTED_EDGE ( 'NONE', *, *, #126017, .F. ) ;
#22241=CARTESIAN_POINT ( 'NONE',  ( -14.59999999999998366, 2.500000000000000000, -0.1000000000000001166 ) ) ;
#22242=ADVANCED_FACE ( 'NONE', ( #4537 ), #82131, .T. ) ;
#22243=LINE ( 'NONE', #50391, #93775 ) ;
#22244=EDGE_CURVE ( 'NONE', #98982, #122996, #38228, .T. ) ;
#22245=EDGE_CURVE ( 'NONE', #71349, #24092, #1984, .T. ) ;
#22246=ORIENTED_EDGE ( 'NONE', *, *, #85992, .T. ) ;
#22247=DIRECTION ( 'NONE',  ( 0.000000000000000000, 1.000000000000000000, 0.000000000000000000 ) ) ;
#22248=CARTESIAN_POINT ( 'NONE',  ( -3.150000000000030109, 12.50000000000000000, 1.883746621131358934 ) ) ;
#22249=AXIS2_PLACEMENT_3D ( 'NONE', #84482, #123735, #22991 ) ;
#22250=AXIS2_PLACEMENT_3D ( 'NONE', #118319, #48953, #116375 ) ;
#22251=EDGE_CURVE ( 'NONE', #95698, #87872, #98838, .T. ) ;
#22252=ORIENTED_EDGE ( 'NONE', *, *, #16265, .T. ) ;
#22253=ADVANCED_FACE ( 'NONE', ( #32119 ), #64131, .T. ) ;
#22254=DIRECTION ( 'NONE',  ( 0.000000000000000000, 1.000000000000000000, 0.000000000000000000 ) ) ;
#22255=EDGE_CURVE ( 'NONE', #34595, #71534, #40377, .T. ) ;
#22256=FACE_OUTER_BOUND ( 'NONE', #114472, .T. ) ;
#22257=AXIS2_PLACEMENT_3D ( 'NONE', #13928, #104259, #102330 ) ;
#22258=AXIS2_PLACEMENT_3D ( 'NONE', #122505, #51194, #32209 ) ;
#22259=ORIENTED_EDGE ( 'NONE', *, *, #14243, .F. ) ;
#22260=AXIS2_PLACEMENT_3D ( 'NONE', #108716, #9880, #49822 ) ;
#22261=DIRECTION ( 'NONE',  ( 0.000000000000000000, 0.000000000000000000, 1.000000000000000000 ) ) ;
#22262=EDGE_CURVE ( 'NONE', #126749, #18676, #51748, .T. ) ;
#22263=LINE ( 'NONE', #79871, #26818 ) ;
#22264=LINE ( 'NONE', #31427, #82822 ) ;
#22265=EDGE_LOOP ( 'NONE', ( #35002, #33247 ) ) ;
#22266=VERTEX_POINT ( 'NONE', #11808 ) ;
#22267=ADVANCED_FACE ( 'NONE', ( #52384 ), #34105, .T. ) ;
#22268=DIRECTION ( 'NONE',  ( -0.000000000000000000, 1.000000000000000000, -0.000000000000000000 ) ) ;
#22269=EDGE_CURVE ( 'NONE', #99205, #52516, #17348, .T. ) ;
#22271=DIRECTION ( 'NONE',  ( -0.000000000000000000, 1.000000000000000000, -0.000000000000000000 ) ) ;
#22272=CARTESIAN_POINT ( 'NONE',  ( -8.350000000000010303, 12.50000000000000000, 6.430097255199259010 ) ) ;
#22273=FACE_OUTER_BOUND ( 'NONE', #85958, .T. ) ;
#22274=ORIENTED_EDGE ( 'NONE', *, *, #110853, .T. ) ;
#22275=FACE_OUTER_BOUND ( 'NONE', #90452, .T. ) ;
#22276=LINE ( 'NONE', #62199, #1727 ) ;
#22277=CARTESIAN_POINT ( 'NONE',  ( -6.650000000000018119, 12.50000000000000000, -7.188010851410854052 ) ) ;
#22278=DIRECTION ( 'NONE',  ( -0.000000000000000000, 1.000000000000000000, -0.000000000000000000 ) ) ;
#22279=LINE ( 'NONE', #53648, #69581 ) ;
#22280=AXIS2_PLACEMENT_3D ( 'NONE', #18209, #117682, #20804 ) ;
#22281=CARTESIAN_POINT ( 'NONE',  ( 10.64999999999990976, 12.50000000000000000, 1.818653347947321475 ) ) ;
#22282=VERTEX_POINT ( 'NONE', #122426 ) ;
#22283=VERTEX_POINT ( 'NONE', #113225 ) ;
#22284=DIRECTION ( 'NONE',  ( 0.000000000000000000, -0.000000000000000000, 1.000000000000000000 ) ) ;
#22285=ORIENTED_EDGE ( 'NONE', *, *, #27456, .F. ) ;
#22286=VECTOR ( 'NONE', #108312, 1000.000000000000000 ) ;
#22287=CIRCLE ( 'NONE', #11794, 0.1000000000000002554 ) ;
#22289=EDGE_LOOP ( 'NONE', ( #53525, #83470 ) ) ;
#22290=VERTEX_POINT ( 'NONE', #14373 ) ;
#22291=AXIS2_PLACEMENT_3D ( 'NONE', #81016, #62026, #20806 ) ;
#22292=ORIENTED_EDGE ( 'NONE', *, *, #34363, .F. ) ;
#22293=DIRECTION ( 'NONE',  ( 0.000000000000000000, 0.000000000000000000, -1.000000000000000000 ) ) ;
#22294=AXIS2_PLACEMENT_3D ( 'NONE', #53142, #3384, #22404 ) ;
#22295=AXIS2_PLACEMENT_3D ( 'NONE', #8044, #127826, #38163 ) ;
#22296=DIRECTION ( 'NONE',  ( 0.000000000000000000, -0.000000000000000000, 1.000000000000000000 ) ) ;
#22297=DIRECTION ( 'NONE',  ( 0.000000000000000000, 0.000000000000000000, 1.000000000000000000 ) ) ;
#22298=AXIS2_PLACEMENT_3D ( 'NONE', #77122, #115743, #27351 ) ;
#22300=PLANE ( 'NONE',  #101674 ) ;
#22301=DIRECTION ( 'NONE',  ( 0.000000000000000000, 0.000000000000000000, -1.000000000000000000 ) ) ;
#22302=DIRECTION ( 'NONE',  ( -4.274815082592931898E-19, -0.9999939076577903929, -0.003490651415223739937 ) ) ;
#22303=CARTESIAN_POINT ( 'NONE',  ( -0.6000000000000388356, 12.50000000000000000, 4.048810130592458201 ) ) ;
#22304=DIRECTION ( 'NONE',  ( 0.000000000000000000, 1.000000000000000000, 0.000000000000000000 ) ) ;
#22305=DIRECTION ( 'NONE',  ( 0.000000000000000000, 1.000000000000000000, 0.000000000000000000 ) ) ;
#22306=AXIS2_PLACEMENT_3D ( 'NONE', #78733, #125866, #28332 ) ;
#22307=ORIENTED_EDGE ( 'NONE', *, *, #87154, .T. ) ;
#22308=EDGE_CURVE ( 'NONE', #48610, #46747, #36267, .T. ) ;
#22309=AXIS2_PLACEMENT_3D ( 'NONE', #27253, #14833, #116276 ) ;
#22310=VECTOR ( 'NONE', #5968, 1000.000000000000000 ) ;
#22311=EDGE_CURVE ( 'NONE', #88940, #59733, #107343, .T. ) ;
#22312=DIRECTION ( 'NONE',  ( -4.274815082592931898E-19, -0.9999939076577903929, -0.003490651415223739937 ) ) ;
#22313=EDGE_LOOP ( 'NONE', ( #109568, #71491, #65358, #59279 ) ) ;
#22314=VERTEX_POINT ( 'NONE', #72676 ) ;
#22315=DIRECTION ( 'NONE',  ( 0.000000000000000000, 1.000000000000000000, 0.000000000000000000 ) ) ;
#22316=DIRECTION ( 'NONE',  ( -0.000000000000000000, -1.000000000000000000, -0.000000000000000000 ) ) ;
#22317=CARTESIAN_POINT ( 'NONE',  ( 8.099999999999921485, 2.500000000000000000, -0.2464101615137783419 ) ) ;
#22318=DIRECTION ( 'NONE',  ( -0.000000000000000000, -1.000000000000000000, -0.000000000000000000 ) ) ;
#22319=DIRECTION ( 'NONE',  ( -0.000000000000000000, 1.000000000000000000, -0.000000000000000000 ) ) ;
#22320=CARTESIAN_POINT ( 'NONE',  ( -10.40000000000000213, 2.500000000000000000, -4.230127018922197557 ) ) ;
#22321=CARTESIAN_POINT ( 'NONE',  ( -6.050000000000020250, 2.500000000000000000, -6.941600689897078347 ) ) ;
#22322=ORIENTED_EDGE ( 'NONE', *, *, #126274, .T. ) ;
#22323=ORIENTED_EDGE ( 'NONE', *, *, #476, .F. ) ;
#22324=ORIENTED_EDGE ( 'NONE', *, *, #118289, .F. ) ;
#22325=ORIENTED_EDGE ( 'NONE', *, *, #4313, .T. ) ;
#22326=VERTEX_POINT ( 'NONE', #33409 ) ;
#22327=CARTESIAN_POINT ( 'NONE',  ( 9.999999999999912959, 2.500000000000000000, 3.637306695894644726 ) ) ;
#22328=CARTESIAN_POINT ( 'NONE',  ( -10.20000000000000284, 2.500000000000000000, -0.3464101615137782364 ) ) ;
#22329=AXIS2_PLACEMENT_3D ( 'NONE', #41275, #2598, #50426 ) ;
#22330=DIRECTION ( 'NONE',  ( -0.000000000000000000, 1.000000000000000000, -0.000000000000000000 ) ) ;
#22331=AXIS2_PLACEMENT_3D ( 'NONE', #16964, #68037, #96846 ) ;
#22332=FACE_OUTER_BOUND ( 'NONE', #63409, .T. ) ;
#22333=DIRECTION ( 'NONE',  ( 0.000000000000000000, 0.000000000000000000, -1.000000000000000000 ) ) ;
#22334=VERTEX_POINT ( 'NONE', #74602 ) ;
#22335=DIRECTION ( 'NONE',  ( 0.000000000000000000, 0.000000000000000000, 1.000000000000000000 ) ) ;
#22336=CARTESIAN_POINT ( 'NONE',  ( 48.83367120242080972, -2.320420704099642517, 5.300559036899318066 ) ) ;
#22337=CARTESIAN_POINT ( 'NONE',  ( 12.69999999999989804, 12.50000000000000000, 0.3464101615137735735 ) ) ;
#22338=CARTESIAN_POINT ( 'NONE',  ( 11.24999999999990763, 12.50000000000000000, -7.188010851410854052 ) ) ;
#22339=CIRCLE ( 'NONE', #68373, 0.06509327318403745899 ) ;
#22340=AXIS2_PLACEMENT_3D ( 'NONE', #70199, #65833, #129147 ) ;
#22341=DIRECTION ( 'NONE',  ( 0.000000000000000000, 1.000000000000000000, 0.000000000000000000 ) ) ;
#22342=EDGE_CURVE ( 'NONE', #66463, #9837, #50930, .T. ) ;
#22343=ORIENTED_EDGE ( 'NONE', *, *, #30915, .F. ) ;
#22344=ORIENTED_EDGE ( 'NONE', *, *, #973, .T. ) ;
#22345=ORIENTED_EDGE ( 'NONE', *, *, #104762, .T. ) ;
#22346=DIRECTION ( 'NONE',  ( 0.000000000000000000, 1.000000000000000000, 0.000000000000000000 ) ) ;
#22347=AXIS2_PLACEMENT_3D ( 'NONE', #23702, #34176, #44631 ) ;
#22348=ORIENTED_EDGE ( 'NONE', *, *, #78930, .T. ) ;
#22349=CIRCLE ( 'NONE', #91284, 0.1000000000000002554 ) ;
#22350=AXIS2_PLACEMENT_3D ( 'NONE', #626, #49762, #70031 ) ;
#22351=DIRECTION ( 'NONE',  ( -0.000000000000000000, -1.000000000000000000, -0.000000000000000000 ) ) ;
#22352=LINE ( 'NONE', #42643, #8463 ) ;
#22353=EDGE_CURVE ( 'NONE', #56590, #92818, #69693, .T. ) ;
#22354=AXIS2_PLACEMENT_3D ( 'NONE', #52646, #2921, #41570 ) ;
#22355=EDGE_CURVE ( 'NONE', #51914, #41353, #48778, .T. ) ;
#22356=ORIENTED_EDGE ( 'NONE', *, *, #43401, .T. ) ;
#22357=CARTESIAN_POINT ( 'NONE',  ( 9.349999999999916156, 2.500000000000000000, 6.941600689897073018 ) ) ;
#22358=CARTESIAN_POINT ( 'NONE',  ( -10.60000000000000142, 2.500000000000000000, -0.2464101615137782308 ) ) ;
#22359=CARTESIAN_POINT ( 'NONE',  ( -7.100000000000013856, 12.50000000000000000, 4.957854068765711553 ) ) ;
#22360=EDGE_CURVE ( 'NONE', #30210, #120000, #107280, .T. ) ;
#22361=CARTESIAN_POINT ( 'NONE',  ( -11.84999999999999609, 12.50000000000000000, 1.818653347947321475 ) ) ;
#22362=CARTESIAN_POINT ( 'NONE',  ( -6.900000000000015454, 12.50000000000000000, 3.918623584224382839 ) ) ;
#22363=ORIENTED_EDGE ( 'NONE', *, *, #50019, .F. ) ;
#22364=ORIENTED_EDGE ( 'NONE', *, *, #114056, .F. ) ;
#22365=EDGE_CURVE ( 'NONE', #114968, #49230, #94732, .T. ) ;
#22367=VECTOR ( 'NONE', #126743, 1000.000000000000000 ) ;
#22368=CARTESIAN_POINT ( 'NONE',  ( -0.2000000000000404232, 12.50000000000000000, 3.983716857408420964 ) ) ;
#22370=DIRECTION ( 'NONE',  ( 0.000000000000000000, 0.000000000000000000, -1.000000000000000000 ) ) ;
#22371=CONICAL_SURFACE ( 'NONE', #74673, 0.09999999999999982514, 0.003490658503988666988 ) ;
#22372=DIRECTION ( 'NONE',  ( -0.000000000000000000, -1.000000000000000000, -0.000000000000000000 ) ) ;
#22373=EDGE_LOOP ( 'NONE', ( #26423, #28835 ) ) ;
#22374=CIRCLE ( 'NONE', #57962, 0.09999999999999982514 ) ;
#22375=EDGE_LOOP ( 'NONE', ( #31992, #68819 ) ) ;
#22376=FACE_OUTER_BOUND ( 'NONE', #102081, .T. ) ;
#22377=LINE ( 'NONE', #43304, #96910 ) ;
#22378=CARTESIAN_POINT ( 'NONE',  ( 2.099999999999950351, 2.500000000000000000, -0.7928203230275542301 ) ) ;
#22379=AXIS2_PLACEMENT_3D ( 'NONE', #111070, #61363, #91453 ) ;
#22380=DIRECTION ( 'NONE',  ( 0.000000000000000000, -0.000000000000000000, 1.000000000000000000 ) ) ;
#22381=ORIENTED_EDGE ( 'NONE', *, *, #80202, .F. ) ;
#22382=CARTESIAN_POINT ( 'NONE',  ( -3.350000000000028511, 12.50000000000000000, 2.922977105672686982 ) ) ;
#22383=VECTOR ( 'NONE', #38785, 1000.000000000000000 ) ;
#22384=DIRECTION ( 'NONE',  ( -0.000000000000000000, 1.000000000000000000, -0.000000000000000000 ) ) ;
#22385=ORIENTED_EDGE ( 'NONE', *, *, #55205, .T. ) ;
#22386=DIRECTION ( 'NONE',  ( 0.000000000000000000, 0.000000000000000000, 1.000000000000000000 ) ) ;
#22387=ORIENTED_EDGE ( 'NONE', *, *, #122862, .F. ) ;
#22388=AXIS2_PLACEMENT_3D ( 'NONE', #74694, #125080, #72123 ) ;
#22389=CARTESIAN_POINT ( 'NONE',  ( -3.350000000000028511, 2.500000000000000000, -1.372243186433550033 ) ) ;
#22390=EDGE_CURVE ( 'NONE', #2669, #125527, #111454, .T. ) ;
#22391=AXIS2_PLACEMENT_3D ( 'NONE', #73927, #115111, #115782 ) ;
#22392=EDGE_LOOP ( 'NONE', ( #113341, #49257 ) ) ;
#22393=LINE ( 'NONE', #53764, #115430 ) ;
#22394=CARTESIAN_POINT ( 'NONE',  ( 0.3999999999999568345, 2.500000000000000000, -3.637306695894650055 ) ) ;
#22395=ORIENTED_EDGE ( 'NONE', *, *, #11140, .F. ) ;
#22396=EDGE_LOOP ( 'NONE', ( #71494, #101925, #64104, #95498 ) ) ;
#22397=ADVANCED_FACE ( 'NONE', ( #65416 ), #78014, .T. ) ;
#22399=LINE ( 'NONE', #62944, #87379 ) ;
#22400=EDGE_CURVE ( 'NONE', #67418, #86712, #13246, .T. ) ;
#22401=FACE_OUTER_BOUND ( 'NONE', #3009, .T. ) ;
#22403=DIRECTION ( 'NONE',  ( 0.000000000000000000, 0.000000000000000000, 1.000000000000000000 ) ) ;
#22404=DIRECTION ( 'NONE',  ( 0.000000000000000000, 0.000000000000000000, 1.000000000000000000 ) ) ;
#22405=DIRECTION ( 'NONE',  ( 0.000000000000000000, -0.9999939076577903929, 0.003490651415223739937 ) ) ;
#22406=EDGE_CURVE ( 'NONE', #28605, #80531, #54955, .T. ) ;
#22407=EDGE_CURVE ( 'NONE', #7993, #45906, #105197, .T. ) ;
#22408=CARTESIAN_POINT ( 'NONE',  ( -7.500000000000016875, 2.500000000000000000, -3.737306695894649700 ) ) ;
#22409=CARTESIAN_POINT ( 'NONE',  ( 13.09999999999990195, 2.500000000000000000, -4.776537180435978414 ) ) ;
#22410=EDGE_CURVE ( 'NONE', #102525, #66158, #11196, .T. ) ;
#22411=VECTOR ( 'NONE', #22760, 1000.000000000000000 ) ;
#22412=EDGE_CURVE ( 'NONE', #12097, #57754, #25781, .T. ) ;
#22413=ORIENTED_EDGE ( 'NONE', *, *, #128966, .T. ) ;
#22414=EDGE_LOOP ( 'NONE', ( #53270, #52441 ) ) ;
#22415=CARTESIAN_POINT ( 'NONE',  ( -10.40000000000000213, 12.50000000000000000, 3.637306695894644726 ) ) ;
#22416=ADVANCED_FACE ( 'NONE', ( #56241 ), #27929, .T. ) ;
#22417=ORIENTED_EDGE ( 'NONE', *, *, #124898, .T. ) ;
#22418=DIRECTION ( 'NONE',  ( 0.000000000000000000, -0.000000000000000000, 1.000000000000000000 ) ) ;
#22419=FACE_OUTER_BOUND ( 'NONE', #95588, .T. ) ;
#22420=CARTESIAN_POINT ( 'NONE',  ( -3.750000000000027534, 12.50000000000000000, 2.857883832488649301 ) ) ;
#22421=ORIENTED_EDGE ( 'NONE', *, *, #103486, .T. ) ;
#22422=ORIENTED_EDGE ( 'NONE', *, *, #84747, .T. ) ;
#22423=FACE_BOUND ( 'NONE', #123725, .T. ) ;
#22424=ORIENTED_EDGE ( 'NONE', *, *, #68680, .T. ) ;
#22425=DIRECTION ( 'NONE',  ( -0.000000000000000000, -1.000000000000000000, -0.000000000000000000 ) ) ;
#22426=FACE_OUTER_BOUND ( 'NONE', #34847, .T. ) ;
#22427=ADVANCED_FACE ( 'NONE', ( #104689 ), #5199, .T. ) ;
#22428=DIRECTION ( 'NONE',  ( 0.000000000000000000, -0.9999939076577903929, 0.003490651415223739937 ) ) ;
#22429=DIRECTION ( 'NONE',  ( 0.000000000000000000, -0.9999939076577903929, 0.003490651415223739937 ) ) ;
#22430=CIRCLE ( 'NONE', #118540, 0.06509327318403745899 ) ;
#22431=DIRECTION ( 'NONE',  ( -0.000000000000000000, 1.000000000000000000, -0.000000000000000000 ) ) ;
#22432=AXIS2_PLACEMENT_3D ( 'NONE', #12964, #52920, #93491 ) ;
#22433=DIRECTION ( 'NONE',  ( -0.000000000000000000, -1.000000000000000000, -0.000000000000000000 ) ) ;
#22434=CARTESIAN_POINT ( 'NONE',  ( -15.79999999999998117, 12.50000000000000000, 0.000000000000000000 ) ) ;
#22435=LINE ( 'NONE', #119969, #19195 ) ;
#22436=DIRECTION ( 'NONE',  ( 0.000000000000000000, 0.000000000000000000, 1.000000000000000000 ) ) ;
#22437=DIRECTION ( 'NONE',  ( 0.000000000000000000, 0.000000000000000000, -1.000000000000000000 ) ) ;
#22438=LINE ( 'NONE', #71507, #38980 ) ;
#22439=AXIS2_PLACEMENT_3D ( 'NONE', #20896, #9139, #60825 ) ;
#22440=VECTOR ( 'NONE', #110540, 1000.000000000000000 ) ;
#22441=ORIENTED_EDGE ( 'NONE', *, *, #31666, .T. ) ;
#22443=VERTEX_POINT ( 'NONE', #126286 ) ;
#22444=DIRECTION ( 'NONE',  ( 0.000000000000000000, 0.000000000000000000, 1.000000000000000000 ) ) ;
#22445=ORIENTED_EDGE ( 'NONE', *, *, #24124, .F. ) ;
#22446=LINE ( 'NONE', #70239, #83163 ) ;
#22447=DIRECTION ( 'NONE',  ( 0.000000000000000000, 1.000000000000000000, 0.000000000000000000 ) ) ;
#22448=VERTEX_POINT ( 'NONE', #67323 ) ;
#22449=ORIENTED_EDGE ( 'NONE', *, *, #72836, .T. ) ;
#22450=ORIENTED_EDGE ( 'NONE', *, *, #49296, .T. ) ;
#22451=DIRECTION ( 'NONE',  ( 0.000000000000000000, 1.000000000000000000, 0.000000000000000000 ) ) ;
#22452=CONICAL_SURFACE ( 'NONE', #91375, 0.09999999999999982514, 0.003490658503988666988 ) ;
#22453=AXIS2_PLACEMENT_3D ( 'NONE', #69552, #111400, #92417 ) ;
#22454=DIRECTION ( 'NONE',  ( 0.000000000000000000, 0.000000000000000000, -1.000000000000000000 ) ) ;
#22455=CARTESIAN_POINT ( 'NONE',  ( -2.900000000000029221, 12.50000000000000000, 0.06509327318403515528 ) ) ;
#22456=DIRECTION ( 'NONE',  ( -0.000000000000000000, -1.000000000000000000, -0.000000000000000000 ) ) ;
#22457=DIRECTION ( 'NONE',  ( 0.000000000000000000, 0.000000000000000000, 1.000000000000000000 ) ) ;
#22458=DIRECTION ( 'NONE',  ( 0.000000000000000000, 0.000000000000000000, 1.000000000000000000 ) ) ;
#22461=VERTEX_POINT ( 'NONE', #77808 ) ;
#22462=AXIS2_PLACEMENT_3D ( 'NONE', #24499, #95813, #26439 ) ;
#22463=EDGE_LOOP ( 'NONE', ( #51362, #101986, #55613, #41326 ) ) ;
#22464=EDGE_CURVE ( 'NONE', #35194, #22628, #82222, .T. ) ;
#22465=EDGE_LOOP ( 'NONE', ( #101232, #5698, #64797, #66986 ) ) ;
#22466=FACE_OUTER_BOUND ( 'NONE', #19643, .T. ) ;
#22467=ORIENTED_EDGE ( 'NONE', *, *, #110254, .F. ) ;
#22468=VERTEX_POINT ( 'NONE', #26152 ) ;
#22470=AXIS2_PLACEMENT_3D ( 'NONE', #72011, #2592, #53010 ) ;
#22471=AXIS2_PLACEMENT_3D ( 'NONE', #80319, #79035, #37806 ) ;
#22473=EDGE_CURVE ( 'NONE', #103996, #48300, #125617, .T. ) ;
#22474=FACE_OUTER_BOUND ( 'NONE', #20928, .T. ) ;
#22475=DIRECTION ( 'NONE',  ( 0.000000000000000000, 0.000000000000000000, 1.000000000000000000 ) ) ;
#22476=AXIS2_PLACEMENT_3D ( 'NONE', #46813, #126661, #76269 ) ;
#22477=DIRECTION ( 'NONE',  ( 0.000000000000000000, 1.000000000000000000, 0.000000000000000000 ) ) ;
#22478=CARTESIAN_POINT ( 'NONE',  ( -1.850000000000033396, 12.50000000000000000, -6.776507416713039689 ) ) ;
#22479=DIRECTION ( 'NONE',  ( 0.000000000000000000, 0.000000000000000000, 1.000000000000000000 ) ) ;
#22480=CIRCLE ( 'NONE', #93554, 0.06509327318403745899 ) ;
#22481=CARTESIAN_POINT ( 'NONE',  ( 14.34999999999989662, 2.500000000000000000, 1.918653347947321564 ) ) ;
#22482=VECTOR ( 'NONE', #27221, 1000.000000000000000 ) ;
#22483=ORIENTED_EDGE ( 'NONE', *, *, #80475, .T. ) ;
#22484=AXIS2_PLACEMENT_3D ( 'NONE', #34723, #3940, #104709 ) ;
#22485=AXIS2_PLACEMENT_3D ( 'NONE', #124408, #24266, #45207 ) ;
#22486=DIRECTION ( 'NONE',  ( 0.000000000000000000, 1.000000000000000000, 0.000000000000000000 ) ) ;
#22487=ORIENTED_EDGE ( 'NONE', *, *, #99399, .F. ) ;
#22488=FACE_OUTER_BOUND ( 'NONE', #37181, .T. ) ;
#22489=ORIENTED_EDGE ( 'NONE', *, *, #128105, .F. ) ;
#22490=DIRECTION ( 'NONE',  ( -0.000000000000000000, -1.000000000000000000, -0.000000000000000000 ) ) ;
#22491=AXIS2_PLACEMENT_3D ( 'NONE', #41773, #51584, #62048 ) ;
#22492=VERTEX_POINT ( 'NONE', #75885 ) ;
#22493=CARTESIAN_POINT ( 'NONE',  ( 10.39999999999991154, 2.500000000000000000, 3.537306695894645081 ) ) ;
#22494=CIRCLE ( 'NONE', #55910, 0.09999999999999999167 ) ;
#22495=AXIS2_PLACEMENT_3D ( 'NONE', #52832, #82950, #16104 ) ;
#22496=DIRECTION ( 'NONE',  ( 0.000000000000000000, 0.000000000000000000, -1.000000000000000000 ) ) ;
#22497=EDGE_LOOP ( 'NONE', ( #108127, #43946 ) ) ;
#22498=ORIENTED_EDGE ( 'NONE', *, *, #126836, .T. ) ;
#22499=DIRECTION ( 'NONE',  ( 0.000000000000000000, -0.9999939076577903929, 0.003490651415223739937 ) ) ;
#22500=FACE_OUTER_BOUND ( 'NONE', #17604, .T. ) ;
#22501=DIRECTION ( 'NONE',  ( 0.000000000000000000, -0.9999939076577903929, 0.003490651415223739937 ) ) ;
#22502=LINE ( 'NONE', #62419, #95290 ) ;
#22503=DIRECTION ( 'NONE',  ( 0.000000000000000000, 1.000000000000000000, 0.000000000000000000 ) ) ;
#22504=ADVANCED_FACE ( 'NONE', ( #66062 ), #96873, .T. ) ;
#22505=ORIENTED_EDGE ( 'NONE', *, *, #97923, .T. ) ;
#22506=DIRECTION ( 'NONE',  ( 0.000000000000000000, -0.9999939076577903929, 0.003490651415223739937 ) ) ;
#22507=AXIS2_PLACEMENT_3D ( 'NONE', #16535, #68872, #27030 ) ;
#22508=ORIENTED_EDGE ( 'NONE', *, *, #1803, .F. ) ;
#22509=FACE_OUTER_BOUND ( 'NONE', #17626, .T. ) ;
#22510=DIRECTION ( 'NONE',  ( -0.000000000000000000, 1.000000000000000000, -0.000000000000000000 ) ) ;
#22511=EDGE_CURVE ( 'NONE', #18296, #81272, #76542, .T. ) ;
#22512=EDGE_CURVE ( 'NONE', #86788, #43040, #57175, .T. ) ;
#22513=ADVANCED_FACE ( 'NONE', ( #86994 ), #42529, .T. ) ;
#22514=DIRECTION ( 'NONE',  ( -0.000000000000000000, -1.000000000000000000, -0.000000000000000000 ) ) ;
#22515=LINE ( 'NONE', #59870, #7079 ) ;
#22516=DIRECTION ( 'NONE',  ( 0.000000000000000000, 0.000000000000000000, 1.000000000000000000 ) ) ;
#22517=DIRECTION ( 'NONE',  ( 0.000000000000000000, -0.9999939076577903929, 0.003490651415223739937 ) ) ;
#22518=EDGE_CURVE ( 'NONE', #77451, #60396, #101087, .T. ) ;
#22520=ORIENTED_EDGE ( 'NONE', *, *, #126109, .F. ) ;
#22521=VECTOR ( 'NONE', #33852, 1000.000000000000000 ) ;
#22522=FACE_OUTER_BOUND ( 'NONE', #21235, .T. ) ;
#22523=AXIS2_PLACEMENT_3D ( 'NONE', #25071, #6058, #74819 ) ;
#22524=DIRECTION ( 'NONE',  ( -0.000000000000000000, -1.000000000000000000, -0.000000000000000000 ) ) ;
#22525=DIRECTION ( 'NONE',  ( 0.000000000000000000, 1.000000000000000000, 0.000000000000000000 ) ) ;
#22526=EDGE_CURVE ( 'NONE', #39789, #119576, #15298, .T. ) ;
#22527=ORIENTED_EDGE ( 'NONE', *, *, #97497, .F. ) ;
#22529=ORIENTED_EDGE ( 'NONE', *, *, #115908, .T. ) ;
#22530=DIRECTION ( 'NONE',  ( 0.000000000000000000, 0.000000000000000000, 1.000000000000000000 ) ) ;
#22531=CIRCLE ( 'NONE', #129432, 0.1000000000000002554 ) ;
#22532=ORIENTED_EDGE ( 'NONE', *, *, #45344, .T. ) ;
#22533=ORIENTED_EDGE ( 'NONE', *, *, #73086, .F. ) ;
#22534=DIRECTION ( 'NONE',  ( 0.000000000000000000, 0.000000000000000000, 1.000000000000000000 ) ) ;
#22535=EDGE_LOOP ( 'NONE', ( #16959, #109650 ) ) ;
#22536=DIRECTION ( 'NONE',  ( 0.000000000000000000, 1.000000000000000000, 0.000000000000000000 ) ) ;
#22537=DIRECTION ( 'NONE',  ( -0.000000000000000000, 1.000000000000000000, -0.000000000000000000 ) ) ;
#22538=CARTESIAN_POINT ( 'NONE',  ( -9.600000000000006750, 12.50000000000000000, -0.7579135962115917113 ) ) ;
#22539=ORIENTED_EDGE ( 'NONE', *, *, #76315, .T. ) ;
#22540=AXIS2_PLACEMENT_3D ( 'NONE', #51711, #13, #80529 ) ;
#22541=FACE_OUTER_BOUND ( 'NONE', #71226, .T. ) ;
#22542=CARTESIAN_POINT ( 'NONE',  ( 8.149999999999920419, 12.50000000000000000, -2.511473670974877948 ) ) ;
#22543=ORIENTED_EDGE ( 'NONE', *, *, #111519, .T. ) ;
#22544=VERTEX_POINT ( 'NONE', #10371 ) ;
#22546=CIRCLE ( 'NONE', #101953, 0.09999999999999982514 ) ;
#22547=DIRECTION ( 'NONE',  ( 0.000000000000000000, 0.000000000000000000, 1.000000000000000000 ) ) ;
#22549=CARTESIAN_POINT ( 'NONE',  ( 10.19999999999991402, 12.50000000000000000, 0.2813168883297361700 ) ) ;
#22550=FACE_BOUND ( 'NONE', #5234, .T. ) ;
#22551=VERTEX_POINT ( 'NONE', #48362 ) ;
#22552=CIRCLE ( 'NONE', #37126, 0.06509327318403741736 ) ;
#22553=CARTESIAN_POINT ( 'NONE',  ( 3.349999999999945466, 2.500000000000000000, -2.957883832488653830 ) ) ;
#22554=CARTESIAN_POINT ( 'NONE',  ( -7.900000000000011013, 2.500000000000000000, 4.230127018922196669 ) ) ;
#22555=AXIS2_PLACEMENT_3D ( 'NONE', #75876, #85051, #105989 ) ;
#22556=ORIENTED_EDGE ( 'NONE', *, *, #81654, .F. ) ;
#22557=CARTESIAN_POINT ( 'NONE',  ( 6.049999999999934097, 12.50000000000000000, 6.148780366869520897 ) ) ;
#22558=CARTESIAN_POINT ( 'NONE',  ( 11.84999999999990372, 2.500000000000000000, -6.148780366869526226 ) ) ;
#22559=VECTOR ( 'NONE', #116672, 1000.000000000000000 ) ;
#22560=LINE ( 'NONE', #64392, #11014 ) ;
#22561=ADVANCED_FACE ( 'NONE', ( #60766 ), #34208, .T. ) ;
#22562=DIRECTION ( 'NONE',  ( 0.000000000000000000, 1.000000000000000000, 0.000000000000000000 ) ) ;
#22563=CARTESIAN_POINT ( 'NONE',  ( -0.6500000000000394351, 2.500000000000000000, 6.841600689897072485 ) ) ;
#22565=DIRECTION ( 'NONE',  ( 0.000000000000000000, 0.000000000000000000, 1.000000000000000000 ) ) ;
#22566=CARTESIAN_POINT ( 'NONE',  ( -12.29999999999999538, 2.500000000000000000, -4.776537180435975749 ) ) ;
#22567=ADVANCED_FACE ( 'NONE', ( #78491 ), #65480, .T. ) ;
#22568=CIRCLE ( 'NONE', #87287, 0.06509327318403745899 ) ;
#22569=EDGE_CURVE ( 'NONE', #39091, #120001, #32062, .T. ) ;
#22570=AXIS2_PLACEMENT_3D ( 'NONE', #9140, #20252, #49088 ) ;
#22571=ORIENTED_EDGE ( 'NONE', *, *, #68573, .T. ) ;
#22572=ORIENTED_EDGE ( 'NONE', *, *, #120553, .F. ) ;
#22573=EDGE_CURVE ( 'NONE', #118322, #100139, #99410, .T. ) ;
#22574=ORIENTED_EDGE ( 'NONE', *, *, #42244, .F. ) ;
#22575=VERTEX_POINT ( 'NONE', #18892 ) ;
#22576=DIRECTION ( 'NONE',  ( -4.274815082592931898E-19, -0.9999939076577903929, -0.003490651415223739937 ) ) ;
#22577=DIRECTION ( 'NONE',  ( -0.000000000000000000, 1.000000000000000000, -0.000000000000000000 ) ) ;
#22578=FACE_OUTER_BOUND ( 'NONE', #121036, .T. ) ;
#22579=CIRCLE ( 'NONE', #10041, 0.09999999999999982514 ) ;
#22580=VERTEX_POINT ( 'NONE', #90864 ) ;
#22581=FACE_BOUND ( 'NONE', #106573, .T. ) ;
#22583=DIRECTION ( 'NONE',  ( 0.000000000000000000, 1.000000000000000000, 0.000000000000000000 ) ) ;
#22584=EDGE_CURVE ( 'NONE', #81852, #113860, #58831, .T. ) ;
#22585=CARTESIAN_POINT ( 'NONE',  ( 4.549999999999937650, 2.500000000000000000, 2.265063509461097357 ) ) ;
#22586=AXIS2_PLACEMENT_3D ( 'NONE', #4712, #103597, #125781 ) ;
#22587=VECTOR ( 'NONE', #48829, 1000.000000000000000 ) ;
#22588=EDGE_CURVE ( 'NONE', #79738, #15950, #19516, .T. ) ;
#22589=LINE ( 'NONE', #82789, #65826 ) ;
#22590=CARTESIAN_POINT ( 'NONE',  ( 0.1999999999999571565, 12.50000000000000000, 3.983716857408420076 ) ) ;
#22591=FACE_OUTER_BOUND ( 'NONE', #100657, .T. ) ;
#22592=FACE_OUTER_BOUND ( 'NONE', #60665, .T. ) ;
#22593=DIRECTION ( 'NONE',  ( 0.000000000000000000, -0.9999939076577903929, 0.003490651415223739937 ) ) ;
#22594=CARTESIAN_POINT ( 'NONE',  ( -7.100000000000014744, 2.500000000000000000, 4.330127018922196314 ) ) ;
#22595=ADVANCED_FACE ( 'NONE', ( #109870 ), #92683, .T. ) ;
#22596=ORIENTED_EDGE ( 'NONE', *, *, #116372, .F. ) ;
#22597=ORIENTED_EDGE ( 'NONE', *, *, #26500, .F. ) ;
#22598=VERTEX_POINT ( 'NONE', #81058 ) ;
#22599=EDGE_LOOP ( 'NONE', ( #62449, #103802, #17418, #22543 ) ) ;
#22600=ORIENTED_EDGE ( 'NONE', *, *, #126836, .F. ) ;
#22602=CARTESIAN_POINT ( 'NONE',  ( -5.600000000000023626, 12.50000000000000000, -4.741630453620015118 ) ) ;
#22604=ORIENTED_EDGE ( 'NONE', *, *, #116704, .T. ) ;
#22605=CARTESIAN_POINT ( 'NONE',  ( -4.150000000000024336, 12.50000000000000000, 2.165063509461097713 ) ) ;
#22606=CARTESIAN_POINT ( 'NONE',  ( 14.69113575703618402, -2.499999999999999556, 6.337000354878961517 ) ) ;
#22607=LINE ( 'NONE', #90675, #45817 ) ;
#22608=FACE_OUTER_BOUND ( 'NONE', #128588, .T. ) ;
#22609=CONICAL_SURFACE ( 'NONE', #118728, 0.09999999999999999167, 0.003490658503988666988 ) ;
#22611=DIRECTION ( 'NONE',  ( 0.000000000000000000, -0.9999939076577903929, 0.003490651415223739937 ) ) ;
#22612=AXIS2_PLACEMENT_3D ( 'NONE', #26312, #55754, #74763 ) ;
#22613=EDGE_LOOP ( 'NONE', ( #68571, #9359 ) ) ;
#22614=AXIS2_PLACEMENT_3D ( 'NONE', #22995, #70793, #23626 ) ;
#22615=VERTEX_POINT ( 'NONE', #129534 ) ;
#22616=DIRECTION ( 'NONE',  ( 0.000000000000000000, 0.000000000000000000, 1.000000000000000000 ) ) ;
#22617=CARTESIAN_POINT ( 'NONE',  ( -2.100000000000034284, 2.500000000000000000, -4.430127018922202176 ) ) ;
#22618=ORIENTED_EDGE ( 'NONE', *, *, #16005, .T. ) ;
#22619=CIRCLE ( 'NONE', #102022, 0.1000000000000002554 ) ;
#22620=VERTEX_POINT ( 'NONE', #49028 ) ;
#22621=DIRECTION ( 'NONE',  ( -4.274815082592931898E-19, -0.9999939076577903929, -0.003490651415223739937 ) ) ;
#22622=EDGE_CURVE ( 'NONE', #85816, #99488, #121934, .T. ) ;
#22623=CONICAL_SURFACE ( 'NONE', #114619, 0.1000000000000000056, 0.003490658503988666988 ) ;
#22624=CARTESIAN_POINT ( 'NONE',  ( 5.649999999999936406, 12.50000000000000000, -6.841600689897077814 ) ) ;
#22625=FACE_OUTER_BOUND ( 'NONE', #92953, .T. ) ;
#22626=CARTESIAN_POINT ( 'NONE',  ( 7.299999999999924327, 2.500000000000000000, 0.4464101615137735513 ) ) ;
#22627=CARTESIAN_POINT ( 'NONE',  ( -13.14999999999999147, 12.50000000000000000, -2.576566944158912964 ) ) ;
#22628=VERTEX_POINT ( 'NONE', #79755 ) ;
#22629=CARTESIAN_POINT ( 'NONE',  ( -0.8500000000000386136, 2.500000000000000000, 2.957883832488649389 ) ) ;
#22630=AXIS2_PLACEMENT_3D ( 'NONE', #57507, #67277, #7091 ) ;
#22631=ORIENTED_EDGE ( 'NONE', *, *, #96520, .F. ) ;
#22632=DIRECTION ( 'NONE',  ( 0.000000000000000000, 0.000000000000000000, 1.000000000000000000 ) ) ;
#22633=CARTESIAN_POINT ( 'NONE',  ( -10.85000000000000142, 2.500000000000000000, -2.065063509461098068 ) ) ;
#22634=DIRECTION ( 'NONE',  ( -0.000000000000000000, -1.000000000000000000, -0.000000000000000000 ) ) ;
#22635=DIRECTION ( 'NONE',  ( -0.000000000000000000, 1.000000000000000000, -0.000000000000000000 ) ) ;
#22636=CARTESIAN_POINT ( 'NONE',  ( 4.149999999999936406, 12.50000000000000000, 6.560283801567334372 ) ) ;
#22637=EDGE_LOOP ( 'NONE', ( #5573, #83462, #124417, #103571 ) ) ;
#22638=LINE ( 'NONE', #52722, #109460 ) ;
#22639=AXIS2_PLACEMENT_3D ( 'NONE', #29401, #16947, #57570 ) ;
#22640=CARTESIAN_POINT ( 'NONE',  ( -13.74999999999998757, 2.500000000000000000, 1.372243186433549367 ) ) ;
#22641=ORIENTED_EDGE ( 'NONE', *, *, #38089, .F. ) ;
#22642=ORIENTED_EDGE ( 'NONE', *, *, #57300, .F. ) ;
#22643=ORIENTED_EDGE ( 'NONE', *, *, #97859, .T. ) ;
#22644=CARTESIAN_POINT ( 'NONE',  ( 2.500000000000002220, 0.9166666666666682950, 10.00000000000000178 ) ) ;
#22645=DIRECTION ( 'NONE',  ( 0.000000000000000000, 0.000000000000000000, 1.000000000000000000 ) ) ;
#22647=AXIS2_PLACEMENT_3D ( 'NONE', #3432, #112755, #83301 ) ;
#22648=CARTESIAN_POINT ( 'NONE',  ( 0.8499999999999557909, 12.50000000000000000, -7.122917578226816815 ) ) ;
#22649=DIRECTION ( 'NONE',  ( 0.000000000000000000, 0.000000000000000000, -1.000000000000000000 ) ) ;
#22650=CIRCLE ( 'NONE', #85417, 0.09999999999999982514 ) ;
#22651=CARTESIAN_POINT ( 'NONE',  ( -14.34999999999998543, 12.50000000000000000, 1.818653347947325472 ) ) ;
#22653=CONICAL_SURFACE ( 'NONE', #18133, 0.1000000000000002554, 0.003490658503988666988 ) ;
#22654=DIRECTION ( 'NONE',  ( 0.000000000000000000, 0.000000000000000000, -1.000000000000000000 ) ) ;
#22655=EDGE_CURVE ( 'NONE', #80727, #116053, #119970, .T. ) ;
#22656=ORIENTED_EDGE ( 'NONE', *, *, #36673, .F. ) ;
#22657=CARTESIAN_POINT ( 'NONE',  ( -9.150000000000009237, 2.500000000000000000, -2.065063509461102065 ) ) ;
#22658=CIRCLE ( 'NONE', #49851, 0.09999999999999982514 ) ;
#22659=ADVANCED_FACE ( 'NONE', ( #120969 ), #86506, .T. ) ;
#22660=CARTESIAN_POINT ( 'NONE',  ( 13.54999999999989591, 2.500000000000000000, -1.918653347947326004 ) ) ;
#22661=DIRECTION ( 'NONE',  ( 0.000000000000000000, -0.000000000000000000, 1.000000000000000000 ) ) ;
#22662=DIRECTION ( 'NONE',  ( 0.000000000000000000, 0.000000000000000000, 1.000000000000000000 ) ) ;
#22663=EDGE_CURVE ( 'NONE', #35730, #79726, #88565, .T. ) ;
#22664=ORIENTED_EDGE ( 'NONE', *, *, #59188, .F. ) ;
#22665=LINE ( 'NONE', #82871, #6893 ) ;
#22666=AXIS2_PLACEMENT_3D ( 'NONE', #110512, #100676, #543 ) ;
#22667=AXIS2_PLACEMENT_3D ( 'NONE', #102821, #74028, #63570 ) ;
#22668=DIRECTION ( 'NONE',  ( -0.000000000000000000, 1.000000000000000000, -0.000000000000000000 ) ) ;
#22669=DIRECTION ( 'NONE',  ( 0.000000000000000000, -0.9999939076577903929, 0.003490651415223739937 ) ) ;
#22671=EDGE_CURVE ( 'NONE', #37370, #11311, #30103, .T. ) ;
#22672=EDGE_CURVE ( 'NONE', #124700, #103089, #69790, .T. ) ;
#22673=EDGE_CURVE ( 'NONE', #26935, #128257, #23824, .T. ) ;
#22674=EDGE_CURVE ( 'NONE', #53806, #6433, #92815, .T. ) ;
#22675=EDGE_CURVE ( 'NONE', #87575, #84227, #44758, .T. ) ;
#22676=ORIENTED_EDGE ( 'NONE', *, *, #67736, .T. ) ;
#22677=DIRECTION ( 'NONE',  ( -0.000000000000000000, -1.000000000000000000, -0.000000000000000000 ) ) ;
#22678=VERTEX_POINT ( 'NONE', #52880 ) ;
#22679=EDGE_LOOP ( 'NONE', ( #35318, #20280, #89017, #49040 ) ) ;
#22680=DIRECTION ( 'NONE',  ( 0.000000000000000000, -0.9999939076577903929, 0.003490651415223739937 ) ) ;
#22681=AXIS2_PLACEMENT_3D ( 'NONE', #1441, #40091, #89823 ) ;
#22682=ADVANCED_FACE ( 'NONE', ( #103273 ), #73793, .T. ) ;
#22683=DIRECTION ( 'NONE',  ( 0.000000000000000000, 0.000000000000000000, -1.000000000000000000 ) ) ;
#22684=CARTESIAN_POINT ( 'NONE',  ( 8.549999999999922551, 2.500000000000000000, -6.248780366869526759 ) ) ;
#22686=ORIENTED_EDGE ( 'NONE', *, *, #115771, .T. ) ;
#22687=AXIS2_PLACEMENT_3D ( 'NONE', #3326, #32809, #51793 ) ;
#22688=CIRCLE ( 'NONE', #85365, 0.06509327318403745899 ) ;
#22689=AXIS2_PLACEMENT_3D ( 'NONE', #55441, #35177, #75712 ) ;
#22690=CARTESIAN_POINT ( 'NONE',  ( 12.09999999999990550, 12.50000000000000000, 3.637306695894644726 ) ) ;
#22692=VERTEX_POINT ( 'NONE', #23400 ) ;
#22693=CARTESIAN_POINT ( 'NONE',  ( -8.300000000000011369, 12.50000000000000000, -0.06509327318403970719 ) ) ;
#22694=DIRECTION ( 'NONE',  ( 0.000000000000000000, 1.000000000000000000, 0.000000000000000000 ) ) ;
#22695=VECTOR ( 'NONE', #54450, 1000.000000000000000 ) ;
#22696=VERTEX_POINT ( 'NONE', #63342 ) ;
#22697=AXIS2_PLACEMENT_3D ( 'NONE', #123680, #64773, #24220 ) ;
#22698=AXIS2_PLACEMENT_3D ( 'NONE', #84486, #34100, #55012 ) ;
#22699=ORIENTED_EDGE ( 'NONE', *, *, #118271, .F. ) ;
#22700=VERTEX_POINT ( 'NONE', #1831 ) ;
#22701=ORIENTED_EDGE ( 'NONE', *, *, #36244, .T. ) ;
#22702=DIRECTION ( 'NONE',  ( 0.000000000000000000, 0.000000000000000000, 1.000000000000000000 ) ) ;
#22703=CARTESIAN_POINT ( 'NONE',  ( 13.12246079397621124, 2.499999999999999556, 7.156134182876439098 ) ) ;
#22704=CARTESIAN_POINT ( 'NONE',  ( -12.09999999999999609, 12.50000000000000000, -0.7579135962115876035 ) ) ;
#22705=FACE_BOUND ( 'NONE', #81587, .T. ) ;
#22706=ORIENTED_EDGE ( 'NONE', *, *, #42342, .T. ) ;
#22708=DIRECTION ( 'NONE',  ( -0.000000000000000000, -1.000000000000000000, -0.000000000000000000 ) ) ;
#22709=CARTESIAN_POINT ( 'NONE',  ( -8.150000000000014566, 2.500000000000000000, -6.841600689897073373 ) ) ;
#22710=CIRCLE ( 'NONE', #116770, 0.1000000000000000056 ) ;
#22711=CARTESIAN_POINT ( 'NONE',  ( -4.800000000000026468, 12.50000000000000000, -4.676537180435978769 ) ) ;
#22712=EDGE_CURVE ( 'NONE', #42689, #27189, #81685, .T. ) ;
#22713=DIRECTION ( 'NONE',  ( 0.000000000000000000, 0.000000000000000000, -1.000000000000000000 ) ) ;
#22714=EDGE_CURVE ( 'NONE', #92990, #51042, #13579, .T. ) ;
#22715=DIRECTION ( 'NONE',  ( 0.000000000000000000, 0.000000000000000000, -1.000000000000000000 ) ) ;
#22716=ADVANCED_FACE ( 'NONE', ( #11657 ), #103245, .T. ) ;
#22717=DIRECTION ( 'NONE',  ( 0.000000000000000000, -0.000000000000000000, 1.000000000000000000 ) ) ;
#22718=ADVANCED_FACE ( 'NONE', ( #62067 ), #15386, .T. ) ;
#22719=EDGE_LOOP ( 'NONE', ( #125222, #124182 ) ) ;
#22720=ORIENTED_EDGE ( 'NONE', *, *, #126690, .T. ) ;
#22721=VERTEX_POINT ( 'NONE', #82997 ) ;
#22722=VECTOR ( 'NONE', #127223, 1000.000000000000000 ) ;
#22723=ORIENTED_EDGE ( 'NONE', *, *, #128803, .T. ) ;
#22724=ORIENTED_EDGE ( 'NONE', *, *, #70364, .T. ) ;
#22725=AXIS2_PLACEMENT_3D ( 'NONE', #21681, #2021, #120524 ) ;
#22726=CARTESIAN_POINT ( 'NONE',  ( 7.099999999999927702, 2.500000000000000000, 4.922947341949748257 ) ) ;
#22727=CARTESIAN_POINT ( 'NONE',  ( -2.100000000000033396, 12.50000000000000000, 0.6928203230275494784 ) ) ;
#22728=EDGE_LOOP ( 'NONE', ( #24457, #122386, #106916, #121313 ) ) ;
#22729=EDGE_CURVE ( 'NONE', #5978, #121861, #34300, .T. ) ;
#22730=FACE_BOUND ( 'NONE', #92334, .T. ) ;
#22731=CARTESIAN_POINT ( 'NONE',  ( 3.149999999999942624, 12.50000000000000000, 6.083687093685483660 ) ) ;
#22732=EDGE_CURVE ( 'NONE', #97422, #51891, #103911, .T. ) ;
#22733=EDGE_CURVE ( 'NONE', #21325, #71846, #105295, .T. ) ;
#22734=ADVANCED_FACE ( 'NONE', ( #122913 ), #122025, .T. ) ;
#22736=ORIENTED_EDGE ( 'NONE', *, *, #117043, .F. ) ;
#22737=DIRECTION ( 'NONE',  ( -0.000000000000000000, -1.000000000000000000, -0.000000000000000000 ) ) ;
#22738=CARTESIAN_POINT ( 'NONE',  ( -0.8500000000000395017, 2.500000000000000000, 6.495190528383297135 ) ) ;
#22739=CARTESIAN_POINT ( 'NONE',  ( -5.600000000000023626, 2.500000000000000000, -4.676537180435977881 ) ) ;
#22740=ORIENTED_EDGE ( 'NONE', *, *, #108916, .T. ) ;
#22741=AXIS2_PLACEMENT_3D ( 'NONE', #86987, #115803, #36625 ) ;
#22742=CARTESIAN_POINT ( 'NONE',  ( 15.59999999999988951, 2.500000000000000000, 0.3464101615137735735 ) ) ;
#22743=EDGE_CURVE ( 'NONE', #16412, #51103, #113708, .T. ) ;
#22744=CIRCLE ( 'NONE', #8134, 0.06509327318403745899 ) ;
#22745=ORIENTED_EDGE ( 'NONE', *, *, #42167, .T. ) ;
#22746=ORIENTED_EDGE ( 'NONE', *, *, #42174, .T. ) ;
#22747=ORIENTED_EDGE ( 'NONE', *, *, #122767, .T. ) ;
#22748=CARTESIAN_POINT ( 'NONE',  ( 11.84999999999990372, 2.500000000000000000, -6.841600689897078702 ) ) ;
#22750=DIRECTION ( 'NONE',  ( -0.000000000000000000, 1.000000000000000000, -0.000000000000000000 ) ) ;
#22751=VECTOR ( 'NONE', #65543, 1000.000000000000000 ) ;
#22752=EDGE_LOOP ( 'NONE', ( #110963, #37650 ) ) ;
#22753=DIRECTION ( 'NONE',  ( 0.000000000000000000, 0.000000000000000000, 1.000000000000000000 ) ) ;
#22754=CARTESIAN_POINT ( 'NONE',  ( 3.549999999999941203, 2.500000000000000000, 6.148780366869520897 ) ) ;
#22755=DIRECTION ( 'NONE',  ( -0.000000000000000000, -1.000000000000000000, -0.000000000000000000 ) ) ;
#22756=AXIS2_PLACEMENT_3D ( 'NONE', #15072, #3357, #73374 ) ;
#22757=DIRECTION ( 'NONE',  ( 0.000000000000000000, -0.000000000000000000, 1.000000000000000000 ) ) ;
#22758=ORIENTED_EDGE ( 'NONE', *, *, #80459, .T. ) ;
#22759=AXIS2_PLACEMENT_3D ( 'NONE', #14786, #82932, #34482 ) ;
#22760=DIRECTION ( 'NONE',  ( -4.274815082592931898E-19, -0.9999939076577903929, -0.003490651415223739937 ) ) ;
#22761=EDGE_CURVE ( 'NONE', #105604, #51184, #61428, .T. ) ;
#22762=ORIENTED_EDGE ( 'NONE', *, *, #96682, .F. ) ;
#22763=CARTESIAN_POINT ( 'NONE',  ( 11.44999999999990514, 2.500000000000000000, 2.511473670974873507 ) ) ;
#22764=AXIS2_PLACEMENT_3D ( 'NONE', #55459, #116294, #67174 ) ;
#22765=CIRCLE ( 'NONE', #83389, 0.1000000000000002554 ) ;
#22766=ORIENTED_EDGE ( 'NONE', *, *, #2043, .T. ) ;
#22768=DIRECTION ( 'NONE',  ( 0.000000000000000000, -0.000000000000000000, 1.000000000000000000 ) ) ;
#22769=DIRECTION ( 'NONE',  ( 0.000000000000000000, 1.000000000000000000, 0.000000000000000000 ) ) ;
#22770=FACE_OUTER_BOUND ( 'NONE', #96068, .T. ) ;
#22771=CARTESIAN_POINT ( 'NONE',  ( 12.69999999999990159, 2.500000000000000000, -4.083716857408426826 ) ) ;
#22772=PLANE ( 'NONE',  #103979 ) ;
#22773=ORIENTED_EDGE ( 'NONE', *, *, #8325, .T. ) ;
#22774=ORIENTED_EDGE ( 'NONE', *, *, #3079, .T. ) ;
#22775=DIRECTION ( 'NONE',  ( 0.000000000000000000, 0.000000000000000000, -1.000000000000000000 ) ) ;
#22776=ADVANCED_FACE ( 'NONE', ( #22793 ), #83635, .T. ) ;
#22777=CARTESIAN_POINT ( 'NONE',  ( 10.64999999999991331, 12.50000000000000000, -2.576566944158915184 ) ) ;
#22778=FACE_OUTER_BOUND ( 'NONE', #68996, .T. ) ;
#22779=VECTOR ( 'NONE', #52977, 1000.000000000000000 ) ;
#22780=VERTEX_POINT ( 'NONE', #71885 ) ;
#22781=ORIENTED_EDGE ( 'NONE', *, *, #124815, .F. ) ;
#22782=CARTESIAN_POINT ( 'NONE',  ( -9.400000000000007461, 12.50000000000000000, 4.676537180435972552 ) ) ;
#22783=VERTEX_POINT ( 'NONE', #111807 ) ;
#22784=CARTESIAN_POINT ( 'NONE',  ( -4.350000000000023626, 12.50000000000000000, -2.511473670974877948 ) ) ;
#22785=FACE_OUTER_BOUND ( 'NONE', #47548, .T. ) ;
#22786=VECTOR ( 'NONE', #125655, 1000.000000000000000 ) ;
#22787=AXIS2_PLACEMENT_3D ( 'NONE', #127910, #38252, #78174 ) ;
#22788=DIRECTION ( 'NONE',  ( -4.274815082592931898E-19, -0.9999939076577903929, -0.003490651415223739937 ) ) ;
#22789=ORIENTED_EDGE ( 'NONE', *, *, #77206, .T. ) ;
#22790=CARTESIAN_POINT ( 'NONE',  ( 13.34999999999990017, 12.50000000000000000, 2.099970236277060032 ) ) ;
#22791=CARTESIAN_POINT ( 'NONE',  ( -4.150000000000028777, 12.50000000000000000, -5.867463478539787225 ) ) ;
#22792=CARTESIAN_POINT ( 'NONE',  ( -1.250000000000035749, 2.500000000000000000, -2.857883832488653741 ) ) ;
#22793=FACE_OUTER_BOUND ( 'NONE', #30913, .T. ) ;
#22794=ADVANCED_FACE ( 'NONE', ( #22151 ), #2464, .T. ) ;
#22795=LINE ( 'NONE', #94726, #41579 ) ;
#22797=ORIENTED_EDGE ( 'NONE', *, *, #79968, .F. ) ;
#22798=VECTOR ( 'NONE', #49031, 1000.000000000000000 ) ;
#22799=AXIS2_PLACEMENT_3D ( 'NONE', #118230, #98564, #77649 ) ;
#22800=DIRECTION ( 'NONE',  ( -0.000000000000000000, 1.000000000000000000, -0.000000000000000000 ) ) ;
#22801=DIRECTION ( 'NONE',  ( 0.000000000000000000, 0.000000000000000000, -1.000000000000000000 ) ) ;
#22802=ORIENTED_EDGE ( 'NONE', *, *, #6834, .T. ) ;
#22803=VERTEX_POINT ( 'NONE', #106484 ) ;
#22805=CARTESIAN_POINT ( 'NONE',  ( 0.8499999999999553468, 12.50000000000000000, 1.472243186433545459 ) ) ;
#22806=LINE ( 'NONE', #1843, #116726 ) ;
#22807=DIRECTION ( 'NONE',  ( 0.000000000000000000, 0.000000000000000000, 1.000000000000000000 ) ) ;
#22808=CARTESIAN_POINT ( 'NONE',  ( -12.89999999999999147, 12.50000000000000000, 5.022947341949748790 ) ) ;
#22809=AXIS2_PLACEMENT_3D ( 'NONE', #2495, #32654, #42461 ) ;
#22810=CARTESIAN_POINT ( 'NONE',  ( 4.149999999999936406, 2.500000000000000000, 6.495190528383297135 ) ) ;
#22811=CARTESIAN_POINT ( 'NONE',  ( 9.149999999999920419, 12.50000000000000000, -5.737276932171712751 ) ) ;
#22812=LINE ( 'NONE', #11675, #74947 ) ;
#22813=DIRECTION ( 'NONE',  ( -0.000000000000000000, 1.000000000000000000, -0.000000000000000000 ) ) ;
#22814=VECTOR ( 'NONE', #50583, 1000.000000000000000 ) ;
#22815=ORIENTED_EDGE ( 'NONE', *, *, #63182, .T. ) ;
#22816=EDGE_LOOP ( 'NONE', ( #35394, #27622 ) ) ;
#22817=EDGE_CURVE ( 'NONE', #12562, #10727, #73998, .T. ) ;
#22818=ORIENTED_EDGE ( 'NONE', *, *, #120326, .F. ) ;
#22819=CIRCLE ( 'NONE', #56140, 0.09999999999999982514 ) ;
#22820=ORIENTED_EDGE ( 'NONE', *, *, #37937, .T. ) ;
#22821=PLANE ( 'NONE',  #88122 ) ;
#22822=CARTESIAN_POINT ( 'NONE',  ( -4.550000000000022915, 12.50000000000000000, 2.165063509461097713 ) ) ;
#22823=ORIENTED_EDGE ( 'NONE', *, *, #118392, .F. ) ;
#22824=DIRECTION ( 'NONE',  ( 0.000000000000000000, 0.000000000000000000, -1.000000000000000000 ) ) ;
#22825=CARTESIAN_POINT ( 'NONE',  ( 9.149999999999918643, 2.500000000000000000, -6.395190528383301931 ) ) ;
#22826=CARTESIAN_POINT ( 'NONE',  ( 12.29999999999990656, 2.500000000000000000, -4.576537180435977348 ) ) ;
#22827=ORIENTED_EDGE ( 'NONE', *, *, #82224, .T. ) ;
#22828=ADVANCED_FACE ( 'NONE', ( #6320 ), #74451, .T. ) ;
#22829=EDGE_CURVE ( 'NONE', #31342, #70284, #51028, .T. ) ;
#22830=ADVANCED_FACE ( 'NONE', ( #44999 ), #9149, .T. ) ;
#22831=CARTESIAN_POINT ( 'NONE',  ( -12.29999999999999538, 2.500000000000000000, 4.676537180435972552 ) ) ;
#22832=EDGE_CURVE ( 'NONE', #69735, #87864, #32159, .T. ) ;
#22833=CIRCLE ( 'NONE', #104289, 0.06509327318403745899 ) ;
#22834=CARTESIAN_POINT ( 'NONE',  ( -0.4500000000000402012, 2.500000000000000000, 6.595190528383296780 ) ) ;
#22835=VERTEX_POINT ( 'NONE', #37112 ) ;
#22836=CIRCLE ( 'NONE', #83472, 0.1000000000000002554 ) ;
#22837=ORIENTED_EDGE ( 'NONE', *, *, #109988, .F. ) ;
#22838=VERTEX_POINT ( 'NONE', #107111 ) ;
#22839=VERTEX_POINT ( 'NONE', #45645 ) ;
#22840=DIRECTION ( 'NONE',  ( -0.000000000000000000, -1.000000000000000000, -0.000000000000000000 ) ) ;
#22841=AXIS2_PLACEMENT_3D ( 'NONE', #110943, #80224, #110320 ) ;
#22842=EDGE_CURVE ( 'NONE', #123328, #100183, #38419, .T. ) ;
#22843=DIRECTION ( 'NONE',  ( 0.000000000000000000, 1.000000000000000000, 0.000000000000000000 ) ) ;
#22844=DIRECTION ( 'NONE',  ( 0.000000000000000000, 0.000000000000000000, -1.000000000000000000 ) ) ;
#22845=EDGE_CURVE ( 'NONE', #117628, #16039, #7624, .T. ) ;
#22846=DIRECTION ( 'NONE',  ( -0.000000000000000000, 1.000000000000000000, -0.000000000000000000 ) ) ;
#22847=ADVANCED_FACE ( 'NONE', ( #75093 ), #101189, .T. ) ;
#22848=EDGE_LOOP ( 'NONE', ( #98458, #84799, #16524, #36367 ) ) ;
#22849=AXIS2_PLACEMENT_3D ( 'NONE', #33447, #111999, #122467 ) ;
#22850=AXIS2_PLACEMENT_3D ( 'NONE', #102681, #54869, #75171 ) ;
#22851=CARTESIAN_POINT ( 'NONE',  ( -4.350000000000023626, 2.500000000000000000, 1.718653347947321386 ) ) ;
#22852=ORIENTED_EDGE ( 'NONE', *, *, #52462, .T. ) ;
#22853=LINE ( 'NONE', #53589, #91456 ) ;
#22854=AXIS2_PLACEMENT_3D ( 'NONE', #67107, #76968, #97246 ) ;
#22855=FACE_OUTER_BOUND ( 'NONE', #123452, .T. ) ;
#22857=ORIENTED_EDGE ( 'NONE', *, *, #99591, .F. ) ;
#22858=CIRCLE ( 'NONE', #110566, 0.06509327318403745899 ) ;
#22859=CONICAL_SURFACE ( 'NONE', #66738, 0.1000000000000000472, 0.003490658503988666988 ) ;
#22860=ORIENTED_EDGE ( 'NONE', *, *, #12365, .F. ) ;
#22861=ORIENTED_EDGE ( 'NONE', *, *, #13016, .F. ) ;
#22862=DIRECTION ( 'NONE',  ( 0.000000000000000000, 1.000000000000000000, 0.000000000000000000 ) ) ;
#22863=DIRECTION ( 'NONE',  ( 0.000000000000000000, 0.000000000000000000, 1.000000000000000000 ) ) ;
#22864=DIRECTION ( 'NONE',  ( 0.000000000000000000, 0.000000000000000000, 1.000000000000000000 ) ) ;
#22865=FACE_BOUND ( 'NONE', #65182, .T. ) ;
#22866=DIRECTION ( 'NONE',  ( 0.000000000000000000, 0.000000000000000000, 1.000000000000000000 ) ) ;
#22867=DIRECTION ( 'NONE',  ( 0.000000000000000000, 0.000000000000000000, -1.000000000000000000 ) ) ;
#22868=DIRECTION ( 'NONE',  ( -0.000000000000000000, -1.000000000000000000, -0.000000000000000000 ) ) ;
#22869=AXIS2_PLACEMENT_3D ( 'NONE', #4183, #126563, #25773 ) ;
#22871=CARTESIAN_POINT ( 'NONE',  ( -6.250000000000017764, 12.50000000000000000, 2.857883832488649301 ) ) ;
#22872=LINE ( 'NONE', #43163, #97119 ) ;
#22874=DIRECTION ( 'NONE',  ( 0.000000000000000000, 0.000000000000000000, 1.000000000000000000 ) ) ;
#22875=ORIENTED_EDGE ( 'NONE', *, *, #46174, .F. ) ;
#22876=VERTEX_POINT ( 'NONE', #35185 ) ;
#22877=DIRECTION ( 'NONE',  ( 0.000000000000000000, 0.000000000000000000, 1.000000000000000000 ) ) ;
#22878=FACE_OUTER_BOUND ( 'NONE', #48524, .T. ) ;
#22879=FACE_BOUND ( 'NONE', #1916, .T. ) ;
#22880=CARTESIAN_POINT ( 'NONE',  ( 2.699999999999944666, 2.500000000000000000, 4.676537180435972552 ) ) ;
#22881=EDGE_CURVE ( 'NONE', #16084, #92620, #124195, .T. ) ;
#22882=ADVANCED_FACE ( 'NONE', ( #65250 ), #78211, .T. ) ;
#22883=ORIENTED_EDGE ( 'NONE', *, *, #60052, .T. ) ;
#22885=DIRECTION ( 'NONE',  ( -4.274815082592931898E-19, -0.9999939076577903929, -0.003490651415223739937 ) ) ;
#22886=CONICAL_SURFACE ( 'NONE', #119019, 0.09999999999999982514, 0.003490658503988666988 ) ;
#22887=ORIENTED_EDGE ( 'NONE', *, *, #42173, .F. ) ;
#22888=DIRECTION ( 'NONE',  ( 0.000000000000000000, 1.000000000000000000, 0.000000000000000000 ) ) ;
#22889=DIRECTION ( 'NONE',  ( 0.000000000000000000, 0.000000000000000000, 1.000000000000000000 ) ) ;
#22890=EDGE_CURVE ( 'NONE', #17735, #98528, #24707, .T. ) ;
#22892=CIRCLE ( 'NONE', #96037, 0.06509327318403745899 ) ;
#22893=EDGE_LOOP ( 'NONE', ( #114673, #125285, #102383, #111829 ) ) ;
#22894=LINE ( 'NONE', #51703, #29792 ) ;
#22895=DIRECTION ( 'NONE',  ( -0.000000000000000000, -1.000000000000000000, -0.000000000000000000 ) ) ;
#22896=EDGE_LOOP ( 'NONE', ( #1937, #124710, #118087, #98008 ) ) ;
#22897=DIRECTION ( 'NONE',  ( 0.000000000000000000, 1.000000000000000000, 0.000000000000000000 ) ) ;
#22898=CARTESIAN_POINT ( 'NONE',  ( -4.200000000000029488, 12.50000000000000000, -4.395220292106239768 ) ) ;
#22899=CARTESIAN_POINT ( 'NONE',  ( -4.800000000000022915, 2.500000000000000000, -0.4464101615137783252 ) ) ;
#22900=AXIS2_PLACEMENT_3D ( 'NONE', #55898, #56539, #85986 ) ;
#22901=ORIENTED_EDGE ( 'NONE', *, *, #26548, .T. ) ;
#22902=EDGE_LOOP ( 'NONE', ( #29509, #125078, #19093, #116108 ) ) ;
#22903=DIRECTION ( 'NONE',  ( 0.000000000000000000, 0.000000000000000000, 1.000000000000000000 ) ) ;
#22904=ORIENTED_EDGE ( 'NONE', *, *, #49435, .T. ) ;
#22905=DIRECTION ( 'NONE',  ( 0.000000000000000000, -0.000000000000000000, 1.000000000000000000 ) ) ;
#22906=PLANE ( 'NONE',  #93298 ) ;
#22907=VERTEX_POINT ( 'NONE', #85551 ) ;
#22908=DIRECTION ( 'NONE',  ( -0.000000000000000000, -1.000000000000000000, -0.000000000000000000 ) ) ;
#22909=CARTESIAN_POINT ( 'NONE',  ( -3.950000000000029932, 2.500000000000000000, -6.248780366869526759 ) ) ;
#22910=CARTESIAN_POINT ( 'NONE',  ( -6.249999999999984901, 2.500000000000000000, -6.595190528383302109 ) ) ;
#22911=LINE ( 'NONE', #51092, #50709 ) ;
#22912=AXIS2_PLACEMENT_3D ( 'NONE', #3455, #92473, #54478 ) ;
#22914=ORIENTED_EDGE ( 'NONE', *, *, #110875, .T. ) ;
#22915=ORIENTED_EDGE ( 'NONE', *, *, #43968, .T. ) ;
#22916=CARTESIAN_POINT ( 'NONE',  ( -8.350000000000008527, 12.50000000000000000, 7.253104124594885960 ) ) ;
#22917=ORIENTED_EDGE ( 'NONE', *, *, #91845, .F. ) ;
#22918=EDGE_CURVE ( 'NONE', #56262, #103079, #77022, .T. ) ;
#22919=FACE_OUTER_BOUND ( 'NONE', #43789, .T. ) ;
#22920=ORIENTED_EDGE ( 'NONE', *, *, #119566, .F. ) ;
#22921=ORIENTED_EDGE ( 'NONE', *, *, #124956, .F. ) ;
#22922=ORIENTED_EDGE ( 'NONE', *, *, #102325, .F. ) ;
#22923=CIRCLE ( 'NONE', #12435, 0.06509327318403741736 ) ;
#22924=CARTESIAN_POINT ( 'NONE',  ( 5.799999999999933209, 12.50000000000000000, -2.385244779468109755E-15 ) ) ;
#22925=CARTESIAN_POINT ( 'NONE',  ( -13.09999999999999254, 2.500000000000000000, 0.3464101615137777923 ) ) ;
#22926=FACE_OUTER_BOUND ( 'NONE', #33681, .T. ) ;
#22927=CONICAL_SURFACE ( 'NONE', #129557, 0.1000000000000002554, 0.003490658503988666988 ) ;
#22928=AXIS2_PLACEMENT_3D ( 'NONE', #65988, #127500, #7050 ) ;
#22929=CARTESIAN_POINT ( 'NONE',  ( -2.900000000000029221, 12.50000000000000000, -2.276824562219559311E-15 ) ) ;
#22931=CARTESIAN_POINT ( 'NONE',  ( -7.100000000000013856, 2.500000000000000000, 3.737306695894644371 ) ) ;
#22932=ADVANCED_FACE ( 'NONE', ( #105189 ), #21780, .T. ) ;
#22933=DIRECTION ( 'NONE',  ( 0.000000000000000000, 1.000000000000000000, 0.000000000000000000 ) ) ;
#22934=DIRECTION ( 'NONE',  ( -0.000000000000000000, -1.000000000000000000, -0.000000000000000000 ) ) ;
#22935=AXIS2_PLACEMENT_3D ( 'NONE', #72316, #33045, #123337 ) ;
#22936=ADVANCED_FACE ( 'NONE', ( #116929 ), #94926, .T. ) ;
#22937=LINE ( 'NONE', #119836, #108354 ) ;
#22938=AXIS2_PLACEMENT_3D ( 'NONE', #2693, #82576, #50512 ) ;
#22939=ORIENTED_EDGE ( 'NONE', *, *, #74667, .F. ) ;
#22940=CARTESIAN_POINT ( 'NONE',  ( -4.550000000000022915, 2.500000000000000000, 6.395190528383296602 ) ) ;
#22941=ORIENTED_EDGE ( 'NONE', *, *, #80921, .F. ) ;
#22942=EDGE_CURVE ( 'NONE', #26576, #80133, #71954, .T. ) ;
#22944=DIRECTION ( 'NONE',  ( 0.000000000000000000, 0.000000000000000000, 1.000000000000000000 ) ) ;
#22945=FACE_OUTER_BOUND ( 'NONE', #26772, .T. ) ;
#22946=DIRECTION ( 'NONE',  ( 0.000000000000000000, 1.000000000000000000, 0.000000000000000000 ) ) ;
#22947=DIRECTION ( 'NONE',  ( -0.000000000000000000, -1.000000000000000000, -0.000000000000000000 ) ) ;
#22948=CARTESIAN_POINT ( 'NONE',  ( -14.39999999999998614, 12.50000000000000000, -0.3464101615137760715 ) ) ;
#22949=CARTESIAN_POINT ( 'NONE',  ( 6.449999999999931788, 2.500000000000000000, -6.048780366869526581 ) ) ;
#22950=LINE ( 'NONE', #94254, #96899 ) ;
#22951=EDGE_LOOP ( 'NONE', ( #127397, #59746, #19976, #20206 ) ) ;
#22952=ORIENTED_EDGE ( 'NONE', *, *, #68195, .T. ) ;
#22953=AXIS2_PLACEMENT_3D ( 'NONE', #20348, #40000, #79907 ) ;
#22954=AXIS2_PLACEMENT_3D ( 'NONE', #35836, #95402, #122935 ) ;
#22955=ORIENTED_EDGE ( 'NONE', *, *, #96702, .T. ) ;
#22956=ADVANCED_FACE ( 'NONE', ( #65906 ), #928, .T. ) ;
#22957=VERTEX_POINT ( 'NONE', #59992 ) ;
#22958=ORIENTED_EDGE ( 'NONE', *, *, #20919, .T. ) ;
#22959=DIRECTION ( 'NONE',  ( 0.000000000000000000, -0.000000000000000000, 1.000000000000000000 ) ) ;
#22960=AXIS2_PLACEMENT_3D ( 'NONE', #103465, #102179, #72084 ) ;
#22961=LINE ( 'NONE', #72704, #104166 ) ;
#22962=VECTOR ( 'NONE', #67686, 1000.000000000000000 ) ;
#22963=EDGE_CURVE ( 'NONE', #59055, #74808, #67843, .T. ) ;
#22964=DIRECTION ( 'NONE',  ( 0.000000000000000000, 0.000000000000000000, -1.000000000000000000 ) ) ;
#22965=CARTESIAN_POINT ( 'NONE',  ( 4.349999999999937472, 12.50000000000000000, 6.841600689897072485 ) ) ;
#22966=CARTESIAN_POINT ( 'NONE',  ( 17.50000000000000000, -0.8333333333333350357, 4.000000000000001776 ) ) ;
#22967=ORIENTED_EDGE ( 'NONE', *, *, #101603, .F. ) ;
#22969=EDGE_CURVE ( 'NONE', #59797, #40211, #113805, .T. ) ;
#22971=CARTESIAN_POINT ( 'NONE',  ( -2.100000000000033840, 2.500000000000000000, 5.022947341949748790 ) ) ;
#22972=ADVANCED_FACE ( 'NONE', ( #129377 ), #15487, .T. ) ;
#22973=CARTESIAN_POINT ( 'NONE',  ( -9.150000000000009237, 12.50000000000000000, -2.792790559304616504 ) ) ;
#22974=ADVANCED_FACE ( 'NONE', ( #117559 ), #21875, .T. ) ;
#22975=DIRECTION ( 'NONE',  ( -0.000000000000000000, 1.000000000000000000, -0.000000000000000000 ) ) ;
#22976=CONICAL_SURFACE ( 'NONE', #56408, 0.09999999999999982514, 0.003490658503988666988 ) ;
#22977=EDGE_LOOP ( 'NONE', ( #16230, #17688, #111061, #123092 ) ) ;
#22978=CONICAL_SURFACE ( 'NONE', #68933, 0.09999999999999982514, 0.003490658503988666988 ) ;
#22979=VERTEX_POINT ( 'NONE', #118884 ) ;
#22980=EDGE_CURVE ( 'NONE', #101321, #22212, #74091, .T. ) ;
#22981=EDGE_LOOP ( 'NONE', ( #69784, #102780 ) ) ;
#22982=CARTESIAN_POINT ( 'NONE',  ( -0.8500000000000390576, 2.500000000000000000, -2.165063509461101710 ) ) ;
#22983=ADVANCED_FACE ( 'NONE', ( #87471 ), #9577, .T. ) ;
#22984=AXIS2_PLACEMENT_3D ( 'NONE', #97523, #16364, #67388 ) ;
#22985=DIRECTION ( 'NONE',  ( 0.000000000000000000, 0.000000000000000000, 1.000000000000000000 ) ) ;
#22986=DIRECTION ( 'NONE',  ( -4.274815082592931898E-19, -0.9999939076577903929, -0.003490651415223739937 ) ) ;
#22987=EDGE_CURVE ( 'NONE', #99389, #81036, #107772, .T. ) ;
#22988=ADVANCED_FACE ( 'NONE', ( #89421 ), #9248, .T. ) ;
#22989=CIRCLE ( 'NONE', #98188, 0.06509327318403745899 ) ;
#22990=ORIENTED_EDGE ( 'NONE', *, *, #50638, .F. ) ;
#22991=DIRECTION ( 'NONE',  ( 0.000000000000000000, 0.000000000000000000, 1.000000000000000000 ) ) ;
#22992=DIRECTION ( 'NONE',  ( 0.000000000000000000, 0.000000000000000000, 1.000000000000000000 ) ) ;
#22993=ADVANCED_FACE ( 'NONE', ( #40336 ), #92883, .T. ) ;
#22994=DIRECTION ( 'NONE',  ( -4.274815082592931898E-19, -0.9999939076577903929, -0.003490651415223739937 ) ) ;
#22995=CARTESIAN_POINT ( 'NONE',  ( -7.500000000000011546, 12.50000000000000000, 3.637306695894644726 ) ) ;
#22996=EDGE_CURVE ( 'NONE', #65538, #75669, #32257, .T. ) ;
#22998=EDGE_LOOP ( 'NONE', ( #68868, #118580, #95255, #90367 ) ) ;
#22999=VERTEX_POINT ( 'NONE', #48208 ) ;
#23000=CARTESIAN_POINT ( 'NONE',  ( 3.949999999999938893, 2.500000000000000000, 6.048780366869520364 ) ) ;
#23001=DIRECTION ( 'NONE',  ( -0.000000000000000000, 1.000000000000000000, -0.000000000000000000 ) ) ;
#23002=CARTESIAN_POINT ( 'NONE',  ( 0.8499999999999527933, 2.500000000000000000, 7.188010851410848723 ) ) ;
#23003=CARTESIAN_POINT ( 'NONE',  ( -12.89999999999999147, 12.50000000000000000, 5.022947341949748790 ) ) ;
#23005=ORIENTED_EDGE ( 'NONE', *, *, #45210, .F. ) ;
#23006=CARTESIAN_POINT ( 'NONE',  ( 3.949999999999940670, 2.500000000000000000, 1.718653347947321386 ) ) ;
#23007=VECTOR ( 'NONE', #108561, 1000.000000000000000 ) ;
#23008=CARTESIAN_POINT ( 'NONE',  ( 11.84999999999990372, 2.500000000000000000, -6.841600689897078702 ) ) ;
#23009=LINE ( 'NONE', #18171, #7940 ) ;
#23010=DIRECTION ( 'NONE',  ( 0.000000000000000000, 0.000000000000000000, 1.000000000000000000 ) ) ;
#23011=ORIENTED_EDGE ( 'NONE', *, *, #111641, .F. ) ;
#23012=CARTESIAN_POINT ( 'NONE',  ( 14.59999999999989484, 2.500000000000000000, 0.5928203230275495006 ) ) ;
#23013=VECTOR ( 'NONE', #46192, 1000.000000000000000 ) ;
#23014=DIRECTION ( 'NONE',  ( 0.000000000000000000, 0.000000000000000000, -1.000000000000000000 ) ) ;
#23015=ORIENTED_EDGE ( 'NONE', *, *, #121374, .T. ) ;
#23016=CARTESIAN_POINT ( 'NONE',  ( -4.600000000000024514, 2.500000000000000000, 0.5928203230275495006 ) ) ;
#23017=ORIENTED_EDGE ( 'NONE', *, *, #56331, .F. ) ;
#23018=DIRECTION ( 'NONE',  ( 0.000000000000000000, 0.000000000000000000, 1.000000000000000000 ) ) ;
#23019=VECTOR ( 'NONE', #101036, 1000.000000000000000 ) ;
#23020=CIRCLE ( 'NONE', #87752, 0.06509327318403745899 ) ;
#23022=EDGE_LOOP ( 'NONE', ( #38633, #25283, #75350 ) ) ;
#23023=FACE_OUTER_BOUND ( 'NONE', #17482, .T. ) ;
#23024=CARTESIAN_POINT ( 'NONE',  ( 12.04999999999990479, 2.500000000000000000, 2.165063509461097713 ) ) ;
#23026=ORIENTED_EDGE ( 'NONE', *, *, #61421, .T. ) ;
#23027=ORIENTED_EDGE ( 'NONE', *, *, #23953, .F. ) ;
#23029=CARTESIAN_POINT ( 'NONE',  ( 11.44999999999990514, 2.500000000000000000, 2.611473670974873151 ) ) ;
#23031=FACE_OUTER_BOUND ( 'NONE', #48661, .T. ) ;
#23032=CARTESIAN_POINT ( 'NONE',  ( 5.849999999999935696, 12.50000000000000000, -7.188010851410854052 ) ) ;
#23033=FACE_OUTER_BOUND ( 'NONE', #123843, .T. ) ;
#23034=CARTESIAN_POINT ( 'NONE',  ( -2.100000000000033396, 12.50000000000000000, -5.022947341949754119 ) ) ;
#23035=DIRECTION ( 'NONE',  ( 0.000000000000000000, 1.000000000000000000, 0.000000000000000000 ) ) ;
#23036=DIRECTION ( 'NONE',  ( 0.000000000000000000, 0.000000000000000000, 1.000000000000000000 ) ) ;
#23037=AXIS2_PLACEMENT_3D ( 'NONE', #65412, #105350, #43228 ) ;
#23038=AXIS2_PLACEMENT_3D ( 'NONE', #75518, #26442, #74896 ) ;
#23039=VERTEX_POINT ( 'NONE', #58680 ) ;
#23040=EDGE_LOOP ( 'NONE', ( #9289, #126682, #50987, #36598 ) ) ;
#23041=LINE ( 'NONE', #81320, #125980 ) ;
#23042=ORIENTED_EDGE ( 'NONE', *, *, #1122, .F. ) ;
#23043=CARTESIAN_POINT ( 'NONE',  ( -9.150000000000005684, 2.500000000000000000, 5.902370205355745192 ) ) ;
#23044=CARTESIAN_POINT ( 'NONE',  ( -12.89999999999999147, 2.500000000000000000, 4.230127018922196669 ) ) ;
#23045=CARTESIAN_POINT ( 'NONE',  ( -4.350000000000023626, 2.500000000000000000, 2.411473670974873862 ) ) ;
#23046=EDGE_LOOP ( 'NONE', ( #50099, #6005, #100450, #13536 ) ) ;
#23047=ORIENTED_EDGE ( 'NONE', *, *, #50173, .T. ) ;
#23048=FACE_BOUND ( 'NONE', #47718, .T. ) ;
#23049=EDGE_LOOP ( 'NONE', ( #48460, #8594 ) ) ;
#23050=DIRECTION ( 'NONE',  ( 0.000000000000000000, 0.000000000000000000, 1.000000000000000000 ) ) ;
#23051=DIRECTION ( 'NONE',  ( 0.000000000000000000, 1.000000000000000000, 0.000000000000000000 ) ) ;
#23052=VECTOR ( 'NONE', #84320, 1000.000000000000000 ) ;
#23053=DIRECTION ( 'NONE',  ( -4.274815082592931898E-19, -0.9999939076577903929, -0.003490651415223739937 ) ) ;
#23054=LINE ( 'NONE', #61704, #84881 ) ;
#23055=DIRECTION ( 'NONE',  ( -0.000000000000000000, -1.000000000000000000, -0.000000000000000000 ) ) ;
#23056=FACE_OUTER_BOUND ( 'NONE', #70508, .T. ) ;
#23057=CARTESIAN_POINT ( 'NONE',  ( 7.499999999999923617, 2.500000000000000000, 0.6928203230275494784 ) ) ;
#23058=DIRECTION ( 'NONE',  ( 0.000000000000000000, 1.000000000000000000, 0.000000000000000000 ) ) ;
#23059=DIRECTION ( 'NONE',  ( 0.000000000000000000, 1.000000000000000000, 0.000000000000000000 ) ) ;
#23060=CARTESIAN_POINT ( 'NONE',  ( -3.749999999999991118, 2.500000000000000000, -2.065063509461102065 ) ) ;
#23061=AXIS2_PLACEMENT_3D ( 'NONE', #9004, #109133, #105453 ) ;
#23062=CARTESIAN_POINT ( 'NONE',  ( 2.099999999999949463, 2.500000000000000000, 0.6928203230275494784 ) ) ;
#23063=AXIS2_PLACEMENT_3D ( 'NONE', #117943, #19082, #120537 ) ;
#23064=EDGE_CURVE ( 'NONE', #73230, #40852, #95027, .T. ) ;
#23065=ORIENTED_EDGE ( 'NONE', *, *, #46746, .T. ) ;
#23066=EDGE_LOOP ( 'NONE', ( #118791, #35039, #81595, #79372 ) ) ;
#23067=AXIS2_PLACEMENT_3D ( 'NONE', #69186, #79667, #8983 ) ;
#23068=EDGE_LOOP ( 'NONE', ( #44440, #51233 ) ) ;
#23069=CARTESIAN_POINT ( 'NONE',  ( 7.949999999999925571, 2.500000000000000000, 2.265063509461097357 ) ) ;
#23070=EDGE_LOOP ( 'NONE', ( #76319, #6008, #32438, #115294 ) ) ;
#23071=DIRECTION ( 'NONE',  ( -0.000000000000000000, -1.000000000000000000, -0.000000000000000000 ) ) ;
#23072=VERTEX_POINT ( 'NONE', #29230 ) ;
#23073=ORIENTED_EDGE ( 'NONE', *, *, #113819, .T. ) ;
#23074=EDGE_LOOP ( 'NONE', ( #116389, #113374 ) ) ;
#23075=CARTESIAN_POINT ( 'NONE',  ( 10.64999999999991331, 2.500000000000000000, -1.818653347947325916 ) ) ;
#23076=CONICAL_SURFACE ( 'NONE', #74, 0.1000000000000002554, 0.003490658503988666988 ) ;
#23077=DIRECTION ( 'NONE',  ( -0.000000000000000000, 1.000000000000000000, -0.000000000000000000 ) ) ;
#23078=DIRECTION ( 'NONE',  ( -0.000000000000000000, -1.000000000000000000, -0.000000000000000000 ) ) ;
#23079=AXIS2_PLACEMENT_3D ( 'NONE', #76628, #116538, #28172 ) ;
#23081=EDGE_CURVE ( 'NONE', #105515, #87409, #90807, .T. ) ;
#23082=DIRECTION ( 'NONE',  ( -0.000000000000000000, 1.000000000000000000, -0.000000000000000000 ) ) ;
#23084=VERTEX_POINT ( 'NONE', #11505 ) ;
#23085=PLANE ( 'NONE',  #41384 ) ;
#23086=ORIENTED_EDGE ( 'NONE', *, *, #109411, .F. ) ;
#23087=VERTEX_POINT ( 'NONE', #50789 ) ;
#23088=EDGE_LOOP ( 'NONE', ( #27769, #59468, #101312, #83603 ) ) ;
#23089=CARTESIAN_POINT ( 'NONE',  ( -4.800000000000024691, 2.500000000000000000, 0.4464101615137735513 ) ) ;
#23090=VERTEX_POINT ( 'NONE', #102466 ) ;
#23091=ADVANCED_FACE ( 'NONE', ( #21992 ), #67819, .T. ) ;
#23092=ORIENTED_EDGE ( 'NONE', *, *, #113086, .F. ) ;
#23093=ORIENTED_EDGE ( 'NONE', *, *, #105284, .F. ) ;
#23095=CARTESIAN_POINT ( 'NONE',  ( -9.200000000000009948, 2.500000000000000000, -4.230127018922197557 ) ) ;
#23097=CARTESIAN_POINT ( 'NONE',  ( -12.09999999999999609, 12.50000000000000000, 4.330127018922196314 ) ) ;
#23098=DIRECTION ( 'NONE',  ( 0.000000000000000000, 0.000000000000000000, -1.000000000000000000 ) ) ;
#23099=AXIS2_PLACEMENT_3D ( 'NONE', #19363, #59985, #59337 ) ;
#23100=CARTESIAN_POINT ( 'NONE',  ( -12.49999999999995914, 12.50000000000000000, 0.06509327318403926310 ) ) ;
#23101=CIRCLE ( 'NONE', #102, 0.06509327318403745899 ) ;
#23102=DIRECTION ( 'NONE',  ( 0.000000000000000000, 0.000000000000000000, 1.000000000000000000 ) ) ;
#23104=DIRECTION ( 'NONE',  ( 0.000000000000000000, 0.000000000000000000, 1.000000000000000000 ) ) ;
#23105=CIRCLE ( 'NONE', #81584, 0.06509327318403745899 ) ;
#23106=ORIENTED_EDGE ( 'NONE', *, *, #104554, .T. ) ;
#23107=ORIENTED_EDGE ( 'NONE', *, *, #1972, .T. ) ;
#23109=DIRECTION ( 'NONE',  ( -0.000000000000000000, -1.000000000000000000, -0.000000000000000000 ) ) ;
#23110=ADVANCED_FACE ( 'NONE', ( #12775 ), #25977, .T. ) ;
#23111=CARTESIAN_POINT ( 'NONE',  ( -14.59999999999998366, 12.50000000000000000, 0.6277270498435143509 ) ) ;
#23113=ORIENTED_EDGE ( 'NONE', *, *, #9371, .F. ) ;
#23114=LINE ( 'NONE', #61772, #20472 ) ;
#23116=ADVANCED_FACE ( 'NONE', ( #33103 ), #111646, .T. ) ;
#23117=DIRECTION ( 'NONE',  ( 0.000000000000000000, 0.000000000000000000, -1.000000000000000000 ) ) ;
#23118=CARTESIAN_POINT ( 'NONE',  ( 0.7999999999999612976, 2.500000000000000000, -1.084202172485504434E-16 ) ) ;
#23119=EDGE_CURVE ( 'NONE', #6508, #77652, #121447, .T. ) ;
#23120=CARTESIAN_POINT ( 'NONE',  ( -8.350000000000012079, 2.500000000000000000, 1.572243186433545548 ) ) ;
#23121=VERTEX_POINT ( 'NONE', #122114 ) ;
#23122=CARTESIAN_POINT ( 'NONE',  ( 2.049999999999948308, 2.500000000000000000, 6.495190528383297135 ) ) ;
#23123=EDGE_CURVE ( 'NONE', #116790, #105625, #126324, .T. ) ;
#23124=EDGE_CURVE ( 'NONE', #110412, #90838, #69884, .T. ) ;
#23125=EDGE_CURVE ( 'NONE', #57799, #7472, #40991, .T. ) ;
#23126=EDGE_LOOP ( 'NONE', ( #67609, #87770 ) ) ;
#23127=FACE_OUTER_BOUND ( 'NONE', #69021, .T. ) ;
#23128=AXIS2_PLACEMENT_3D ( 'NONE', #126473, #106809, #17786 ) ;
#23129=DIRECTION ( 'NONE',  ( -0.000000000000000000, -1.000000000000000000, -0.000000000000000000 ) ) ;
#23130=AXIS2_PLACEMENT_3D ( 'NONE', #33868, #6317, #38410 ) ;
#23131=EDGE_CURVE ( 'NONE', #109488, #19106, #92643, .T. ) ;
#23133=CARTESIAN_POINT ( 'NONE',  ( 3.749999999999940492, 2.500000000000000000, 2.857883832488649301 ) ) ;
#23134=CARTESIAN_POINT ( 'NONE',  ( -0.8500000000000382805, 2.500000000000000000, -7.288010851410854585 ) ) ;
#23135=CARTESIAN_POINT ( 'NONE',  ( 12.49999999999990052, 12.50000000000000000, 0.7579135962115869374 ) ) ;
#23136=LINE ( 'NONE', #126500, #20356 ) ;
#23137=EDGE_LOOP ( 'NONE', ( #125394, #108303, #81718, #61051 ) ) ;
#23138=AXIS2_PLACEMENT_3D ( 'NONE', #122173, #59401, #90101 ) ;
#23139=EDGE_CURVE ( 'NONE', #90522, #99720, #122748, .T. ) ;
#23140=DIRECTION ( 'NONE',  ( 0.000000000000000000, 1.000000000000000000, 0.000000000000000000 ) ) ;
#23141=CARTESIAN_POINT ( 'NONE',  ( -11.64999999999999858, 2.500000000000000000, -1.472243186433546125 ) ) ;
#23142=DIRECTION ( 'NONE',  ( 0.000000000000000000, -0.000000000000000000, 1.000000000000000000 ) ) ;
#23143=EDGE_LOOP ( 'NONE', ( #32782, #35104 ) ) ;
#23144=DIRECTION ( 'NONE',  ( -4.274815082592931898E-19, -0.9999939076577903929, -0.003490651415223739937 ) ) ;
#23145=CIRCLE ( 'NONE', #37821, 0.06509327318403743123 ) ;
#23146=VECTOR ( 'NONE', #62623, 1000.000000000000000 ) ;
#23147=ORIENTED_EDGE ( 'NONE', *, *, #16123, .T. ) ;
#23148=ORIENTED_EDGE ( 'NONE', *, *, #23886, .T. ) ;
#23149=DIRECTION ( 'NONE',  ( 0.000000000000000000, 0.000000000000000000, -1.000000000000000000 ) ) ;
#23150=EDGE_LOOP ( 'NONE', ( #26321, #107768 ) ) ;
#23151=CARTESIAN_POINT ( 'NONE',  ( 21.15177371151418839, -2.593223176056361545, -4.151029080743455779 ) ) ;
#23152=CARTESIAN_POINT ( 'NONE',  ( 9.799999999999915445, 12.50000000000000000, -4.611443907251939756 ) ) ;
#23153=CARTESIAN_POINT ( 'NONE',  ( 13.74999999999989519, 2.500000000000000000, -2.857883832488653741 ) ) ;
#23154=ORIENTED_EDGE ( 'NONE', *, *, #53439, .T. ) ;
#23155=DIRECTION ( 'NONE',  ( 0.000000000000000000, 0.000000000000000000, 1.000000000000000000 ) ) ;
#23156=CARTESIAN_POINT ( 'NONE',  ( 6.449999999999930012, 2.500000000000000000, 1.818653347947321475 ) ) ;
#23157=CIRCLE ( 'NONE', #90051, 0.09999999999999982514 ) ;
#23158=ORIENTED_EDGE ( 'NONE', *, *, #71138, .F. ) ;
#23159=EDGE_CURVE ( 'NONE', #251, #51891, #13435, .T. ) ;
#23160=VERTEX_POINT ( 'NONE', #1671 ) ;
#23161=ORIENTED_EDGE ( 'NONE', *, *, #96226, .F. ) ;
#23162=CARTESIAN_POINT ( 'NONE',  ( 0.3999999999999628852, 12.50000000000000000, 0.6928203230275518099 ) ) ;
#23163=CARTESIAN_POINT ( 'NONE',  ( 14.79999999999989235, 2.500000000000000000, 0.4464101615137735513 ) ) ;
#23164=DIRECTION ( 'NONE',  ( 0.000000000000000000, 0.000000000000000000, 1.000000000000000000 ) ) ;
#23166=CARTESIAN_POINT ( 'NONE',  ( -13.29999999999999005, 12.50000000000000000, 0.06509327318403926310 ) ) ;
#23167=DIRECTION ( 'NONE',  ( 0.000000000000000000, 0.000000000000000000, -1.000000000000000000 ) ) ;
#23168=EDGE_LOOP ( 'NONE', ( #95211, #5511, #51101, #79071 ) ) ;
#23169=EDGE_CURVE ( 'NONE', #38948, #32144, #101824, .T. ) ;
#23170=DIRECTION ( 'NONE',  ( 0.000000000000000000, -0.000000000000000000, 1.000000000000000000 ) ) ;
#23171=CARTESIAN_POINT ( 'NONE',  ( 6.049999999999934097, 2.500000000000000000, -2.511473670974877948 ) ) ;
#23172=CIRCLE ( 'NONE', #79622, 0.1000000000000002554 ) ;
#23173=CARTESIAN_POINT ( 'NONE',  ( 5.399999999999932854, 2.500000000000000000, 3.537306695894645081 ) ) ;
#23175=CARTESIAN_POINT ( 'NONE',  ( 10.39999999999991154, 2.500000000000000000, 5.122947341949749323 ) ) ;
#23176=AXIS2_PLACEMENT_3D ( 'NONE', #25676, #25041, #26337 ) ;
#23177=AXIS2_PLACEMENT_3D ( 'NONE', #122104, #120802, #32458 ) ;
#23178=DIRECTION ( 'NONE',  ( 0.000000000000000000, 0.000000000000000000, -1.000000000000000000 ) ) ;
#23179=CARTESIAN_POINT ( 'NONE',  ( 0.5999999999999555689, 2.500000000000000000, 4.776537180435972196 ) ) ;
#23180=AXIS2_PLACEMENT_3D ( 'NONE', #37487, #65632, #116022 ) ;
#23182=EDGE_LOOP ( 'NONE', ( #64573, #106870, #82671, #84405 ) ) ;
#23183=VERTEX_POINT ( 'NONE', #3619 ) ;
#23184=ORIENTED_EDGE ( 'NONE', *, *, #66351, .T. ) ;
#23185=CARTESIAN_POINT ( 'NONE',  ( -12.04999999999999538, 2.500000000000000000, 6.495190528383297135 ) ) ;
#23186=FACE_OUTER_BOUND ( 'NONE', #70334, .T. ) ;
#23187=CONICAL_SURFACE ( 'NONE', #127751, 0.1000000000000002554, 0.003490658503988666988 ) ;
#23188=CARTESIAN_POINT ( 'NONE',  ( -12.09999999999999609, 2.500000000000000000, -0.7928203230275502333 ) ) ;
#23189=EDGE_LOOP ( 'NONE', ( #108998, #125554 ) ) ;
#23190=FACE_BOUND ( 'NONE', #73569, .T. ) ;
#23191=FACE_OUTER_BOUND ( 'NONE', #127704, .T. ) ;
#23192=CARTESIAN_POINT ( 'NONE',  ( -11.64999999999999680, 2.500000000000000000, 1.572243186433545548 ) ) ;
#23193=DIRECTION ( 'NONE',  ( -0.000000000000000000, 1.000000000000000000, -0.000000000000000000 ) ) ;
#23194=LINE ( 'NONE', #50729, #120221 ) ;
#23195=CARTESIAN_POINT ( 'NONE',  ( 2.099999999999949463, 2.500000000000000000, -3.737306695894649700 ) ) ;
#23196=CARTESIAN_POINT ( 'NONE',  ( 7.299999999999926104, 2.500000000000000000, -0.4464101615137782142 ) ) ;
#23197=CARTESIAN_POINT ( 'NONE',  ( 6.249999999999932498, 12.50000000000000000, -2.857883832488653741 ) ) ;
#23198=DIRECTION ( 'NONE',  ( 0.000000000000000000, 1.000000000000000000, 0.000000000000000000 ) ) ;
#23199=CARTESIAN_POINT ( 'NONE',  ( -11.89999999999999680, 2.500000000000000000, 0.4464101615137776591 ) ) ;
#23200=VERTEX_POINT ( 'NONE', #93290 ) ;
#23201=EDGE_CURVE ( 'NONE', #49883, #34238, #30193, .T. ) ;
#23202=CIRCLE ( 'NONE', #35736, 0.09999999999999982514 ) ;
#23203=ORIENTED_EDGE ( 'NONE', *, *, #114857, .F. ) ;
#23204=EDGE_LOOP ( 'NONE', ( #83516, #95039, #70400, #15803 ) ) ;
#23205=ORIENTED_EDGE ( 'NONE', *, *, #22113, .F. ) ;
#23206=ORIENTED_EDGE ( 'NONE', *, *, #113177, .T. ) ;
#23207=ORIENTED_EDGE ( 'NONE', *, *, #66433, .F. ) ;
#23208=CARTESIAN_POINT ( 'NONE',  ( 9.399999999999915090, 12.50000000000000000, 3.983716857408420964 ) ) ;
#23209=ORIENTED_EDGE ( 'NONE', *, *, #9792, .F. ) ;
#23210=EDGE_LOOP ( 'NONE', ( #52948, #5984 ) ) ;
#23211=AXIS2_PLACEMENT_3D ( 'NONE', #43259, #125647, #73330 ) ;
#23212=EDGE_CURVE ( 'NONE', #33523, #91737, #103344, .T. ) ;
#23213=CIRCLE ( 'NONE', #27406, 0.1000000000000000472 ) ;
#23214=DIRECTION ( 'NONE',  ( -0.000000000000000000, 1.000000000000000000, -0.000000000000000000 ) ) ;
#23215=LINE ( 'NONE', #44153, #85513 ) ;
#23216=DIRECTION ( 'NONE',  ( -0.000000000000000000, -1.000000000000000000, -0.000000000000000000 ) ) ;
#23217=ADVANCED_FACE ( 'NONE', ( #113576 ), #23915, .T. ) ;
#23218=EDGE_CURVE ( 'NONE', #71153, #79916, #76144, .T. ) ;
#23219=ORIENTED_EDGE ( 'NONE', *, *, #102902, .T. ) ;
#23220=DIRECTION ( 'NONE',  ( 0.000000000000000000, 1.000000000000000000, 0.000000000000000000 ) ) ;
#23221=VECTOR ( 'NONE', #116509, 1000.000000000000000 ) ;
#23222=AXIS2_PLACEMENT_3D ( 'NONE', #15839, #45969, #85859 ) ;
#23223=VERTEX_POINT ( 'NONE', #41639 ) ;
#23224=ORIENTED_EDGE ( 'NONE', *, *, #1260, .T. ) ;
#23225=PLANE ( 'NONE',  #59363 ) ;
#23226=EDGE_CURVE ( 'NONE', #23494, #87229, #120062, .T. ) ;
#23227=DIRECTION ( 'NONE',  ( 0.000000000000000000, 0.000000000000000000, 1.000000000000000000 ) ) ;
#23228=EDGE_CURVE ( 'NONE', #114181, #69451, #63723, .T. ) ;
#23229=EDGE_LOOP ( 'NONE', ( #64461, #111297 ) ) ;
#23230=ORIENTED_EDGE ( 'NONE', *, *, #63892, .F. ) ;
#23231=AXIS2_PLACEMENT_3D ( 'NONE', #97994, #99943, #50209 ) ;
#23232=CARTESIAN_POINT ( 'NONE',  ( -2.499999999999996447, 12.50000000000000000, 4.395220292106234439 ) ) ;
#23233=VECTOR ( 'NONE', #118147, 1000.000000000000000 ) ;
#23234=DIRECTION ( 'NONE',  ( 0.000000000000000000, 0.000000000000000000, 1.000000000000000000 ) ) ;
#23235=CARTESIAN_POINT ( 'NONE',  ( 9.149999999999916866, 2.500000000000000000, 7.288010851410849256 ) ) ;
#23236=DIRECTION ( 'NONE',  ( -0.000000000000000000, -1.000000000000000000, -0.000000000000000000 ) ) ;
#23237=DIRECTION ( 'NONE',  ( -4.274815082592931898E-19, -0.9999939076577903929, -0.003490651415223739937 ) ) ;
#23238=CIRCLE ( 'NONE', #98625, 0.06509327318403745899 ) ;
#23239=ORIENTED_EDGE ( 'NONE', *, *, #30549, .F. ) ;
#23240=CARTESIAN_POINT ( 'NONE',  ( 3.677302434130775843, -2.499999999999999556, 9.000000000000007105 ) ) ;
#23241=VERTEX_POINT ( 'NONE', #76875 ) ;
#23242=CARTESIAN_POINT ( 'NONE',  ( 1.249999999999988454, 12.50000000000000000, -2.230156782645139391 ) ) ;
#23243=VERTEX_POINT ( 'NONE', #15998 ) ;
#23244=CARTESIAN_POINT ( 'NONE',  ( 8.349999999999923261, 2.500000000000000000, 2.957883832488649389 ) ) ;
#23245=CIRCLE ( 'NONE', #96399, 0.06509327318403745899 ) ;
#23246=CARTESIAN_POINT ( 'NONE',  ( -8.150000000000012790, 12.50000000000000000, 1.818653347947321475 ) ) ;
#23247=LINE ( 'NONE', #73636, #21561 ) ;
#23248=CARTESIAN_POINT ( 'NONE',  ( -10.45000000000000107, 12.50000000000000000, 6.495190528383297135 ) ) ;
#23249=ORIENTED_EDGE ( 'NONE', *, *, #21896, .F. ) ;
#23250=DIRECTION ( 'NONE',  ( -0.000000000000000000, 1.000000000000000000, -0.000000000000000000 ) ) ;
#23251=CARTESIAN_POINT ( 'NONE',  ( -3.749999999999994671, 2.500000000000000000, -6.395190528383301931 ) ) ;
#23252=ORIENTED_EDGE ( 'NONE', *, *, #13615, .F. ) ;
#23253=VERTEX_POINT ( 'NONE', #114221 ) ;
#23254=ORIENTED_EDGE ( 'NONE', *, *, #63387, .F. ) ;
#23255=CARTESIAN_POINT ( 'NONE',  ( -7.050000000000016698, 12.50000000000000000, -6.495190528383302464 ) ) ;
#23256=CARTESIAN_POINT ( 'NONE',  ( 2.949999999999946887, 12.50000000000000000, -2.099970236277064473 ) ) ;
#23258=DIRECTION ( 'NONE',  ( -0.000000000000000000, -1.000000000000000000, -0.000000000000000000 ) ) ;
#23259=DIRECTION ( 'NONE',  ( 0.000000000000000000, -0.000000000000000000, 1.000000000000000000 ) ) ;
#23260=EDGE_CURVE ( 'NONE', #16038, #39771, #92971, .T. ) ;
#23261=DIRECTION ( 'NONE',  ( 0.000000000000000000, 0.000000000000000000, 1.000000000000000000 ) ) ;
#23262=DIRECTION ( 'NONE',  ( -0.000000000000000000, -1.000000000000000000, -0.000000000000000000 ) ) ;
#23263=AXIS2_PLACEMENT_3D ( 'NONE', #128896, #50311, #18265 ) ;
#23264=ADVANCED_FACE ( 'NONE', ( #105694 ), #76245, .T. ) ;
#23265=AXIS2_PLACEMENT_3D ( 'NONE', #111302, #80591, #93467 ) ;
#23266=EDGE_CURVE ( 'NONE', #21207, #49328, #51206, .T. ) ;
#23267=CIRCLE ( 'NONE', #27461, 0.06509327318403745899 ) ;
#23268=ADVANCED_FACE ( 'NONE', ( #56568 ), #116781, .T. ) ;
#23269=ADVANCED_FACE ( 'NONE', ( #125326 ), #86699, .T. ) ;
#23270=ORIENTED_EDGE ( 'NONE', *, *, #45543, .F. ) ;
#23271=DIRECTION ( 'NONE',  ( 0.000000000000000000, 1.000000000000000000, 0.000000000000000000 ) ) ;
#23272=CONICAL_SURFACE ( 'NONE', #110995, 0.1000000000000002554, 0.003490658503988666988 ) ;
#23273=AXIS2_PLACEMENT_3D ( 'NONE', #78948, #88751, #27894 ) ;
#23274=ORIENTED_EDGE ( 'NONE', *, *, #126373, .T. ) ;
#23275=ADVANCED_FACE ( 'NONE', ( #96488 ), #116141, .T. ) ;
#23276=DIRECTION ( 'NONE',  ( 0.000000000000000000, 1.000000000000000000, 0.000000000000000000 ) ) ;
#23277=AXIS2_PLACEMENT_3D ( 'NONE', #37585, #8102, #88606 ) ;
#23278=CARTESIAN_POINT ( 'NONE',  ( 3.749999999999978684, 12.50000000000000000, -6.495190528383302464 ) ) ;
#23279=CARTESIAN_POINT ( 'NONE',  ( 15.59999999999988951, 12.50000000000000000, 0.3464101615137735735 ) ) ;
#23280=CARTESIAN_POINT ( 'NONE',  ( -12.04999999999999538, 2.500000000000000000, 6.395190528383296602 ) ) ;
#23281=ORIENTED_EDGE ( 'NONE', *, *, #57066, .F. ) ;
#23282=ADVANCED_FACE ( 'NONE', ( #6178 ), #85399, .T. ) ;
#23283=DIRECTION ( 'NONE',  ( 0.000000000000000000, 0.000000000000000000, -1.000000000000000000 ) ) ;
#23284=EDGE_CURVE ( 'NONE', #22957, #52516, #75571, .T. ) ;
#23285=DIRECTION ( 'NONE',  ( 0.000000000000000000, 0.000000000000000000, 1.000000000000000000 ) ) ;
#23286=CARTESIAN_POINT ( 'NONE',  ( -13.09999999999999076, 2.500000000000000000, 4.676537180435972552 ) ) ;
#23287=ORIENTED_EDGE ( 'NONE', *, *, #97921, .T. ) ;
#23288=EDGE_LOOP ( 'NONE', ( #25190, #124669 ) ) ;
#23289=CARTESIAN_POINT ( 'NONE',  ( -11.05000000000000071, 12.50000000000000000, -6.841600689897075149 ) ) ;
#23290=ORIENTED_EDGE ( 'NONE', *, *, #27220, .F. ) ;
#23291=ORIENTED_EDGE ( 'NONE', *, *, #25058, .T. ) ;
#23292=CARTESIAN_POINT ( 'NONE',  ( 4.149999999999939959, 2.500000000000000000, -6.595190528383302109 ) ) ;
#23293=EDGE_LOOP ( 'NONE', ( #89900, #105828 ) ) ;
#23294=FACE_OUTER_BOUND ( 'NONE', #91185, .T. ) ;
#23296=DIRECTION ( 'NONE',  ( -0.000000000000000000, 1.000000000000000000, -0.000000000000000000 ) ) ;
#23297=AXIS2_PLACEMENT_3D ( 'NONE', #107804, #57422, #58073 ) ;
#23298=ORIENTED_EDGE ( 'NONE', *, *, #47184, .F. ) ;
#23299=CIRCLE ( 'NONE', #67189, 0.06509327318403741736 ) ;
#23300=CARTESIAN_POINT ( 'NONE',  ( -12.69999999999999396, 2.500000000000000000, -3.983716857408423628 ) ) ;
#23302=ORIENTED_EDGE ( 'NONE', *, *, #62126, .F. ) ;
#23303=DIRECTION ( 'NONE',  ( 0.000000000000000000, 0.000000000000000000, -1.000000000000000000 ) ) ;
#23304=CARTESIAN_POINT ( 'NONE',  ( 13.09999999999990195, 12.50000000000000000, -4.676537180435978769 ) ) ;
#23305=AXIS2_PLACEMENT_3D ( 'NONE', #100110, #78550, #117781 ) ;
#23307=CIRCLE ( 'NONE', #58835, 0.1000000000000002554 ) ;
#23308=ORIENTED_EDGE ( 'NONE', *, *, #16745, .T. ) ;
#23309=ORIENTED_EDGE ( 'NONE', *, *, #117179, .F. ) ;
#23310=VERTEX_POINT ( 'NONE', #84761 ) ;
#23311=CARTESIAN_POINT ( 'NONE',  ( 9.599999999999917932, 12.50000000000000000, 0.6928203230275494784 ) ) ;
#23312=DIRECTION ( 'NONE',  ( -0.000000000000000000, 1.000000000000000000, -0.000000000000000000 ) ) ;
#23313=FACE_OUTER_BOUND ( 'NONE', #97924, .T. ) ;
#23314=FACE_BOUND ( 'NONE', #99131, .T. ) ;
#23315=ORIENTED_EDGE ( 'NONE', *, *, #39993, .T. ) ;
#23317=DIRECTION ( 'NONE',  ( -0.000000000000000000, -1.000000000000000000, -0.000000000000000000 ) ) ;
#23318=DIRECTION ( 'NONE',  ( -0.000000000000000000, -1.000000000000000000, -0.000000000000000000 ) ) ;
#23319=AXIS2_PLACEMENT_3D ( 'NONE', #95279, #84150, #4937 ) ;
#23320=CIRCLE ( 'NONE', #121618, 0.06509327318403745899 ) ;
#23321=ADVANCED_FACE ( 'NONE', ( #115480 ), #126415, .T. ) ;
#23322=AXIS2_PLACEMENT_3D ( 'NONE', #23286, #33756, #2341 ) ;
#23323=DIRECTION ( 'NONE',  ( -0.000000000000000000, 1.000000000000000000, -0.000000000000000000 ) ) ;
#23324=CARTESIAN_POINT ( 'NONE',  ( 1.449999999999951328, 2.500000000000000000, -1.918653347947326004 ) ) ;
#23325=DIRECTION ( 'NONE',  ( 0.000000000000000000, 0.000000000000000000, 1.000000000000000000 ) ) ;
#23326=FACE_OUTER_BOUND ( 'NONE', #112588, .T. ) ;
#23327=EDGE_LOOP ( 'NONE', ( #83420, #115432 ) ) ;
#23328=CONICAL_SURFACE ( 'NONE', #56765, 0.1000000000000002554, 0.003490658503988666988 ) ;
#23329=EDGE_LOOP ( 'NONE', ( #95494, #74256, #109179, #105615 ) ) ;
#23330=ORIENTED_EDGE ( 'NONE', *, *, #124898, .F. ) ;
#23331=ORIENTED_EDGE ( 'NONE', *, *, #58709, .F. ) ;
#23332=ORIENTED_EDGE ( 'NONE', *, *, #100635, .T. ) ;
#23333=CARTESIAN_POINT ( 'NONE',  ( 13.74999999999993427, 2.500000000000000000, 2.265063509461097357 ) ) ;
#23334=DIRECTION ( 'NONE',  ( 0.000000000000000000, 0.000000000000000000, 1.000000000000000000 ) ) ;
#23335=ORIENTED_EDGE ( 'NONE', *, *, #53121, .T. ) ;
#23336=FACE_BOUND ( 'NONE', #66947, .T. ) ;
#23337=DIRECTION ( 'NONE',  ( 0.000000000000000000, 1.000000000000000000, 0.000000000000000000 ) ) ;
#23338=ORIENTED_EDGE ( 'NONE', *, *, #108181, .F. ) ;
#23339=DIRECTION ( 'NONE',  ( 0.000000000000000000, 0.000000000000000000, -1.000000000000000000 ) ) ;
#23340=DIRECTION ( 'NONE',  ( 0.000000000000000000, 1.000000000000000000, 0.000000000000000000 ) ) ;
#23341=DIRECTION ( 'NONE',  ( 0.000000000000000000, 0.000000000000000000, -1.000000000000000000 ) ) ;
#23342=ORIENTED_EDGE ( 'NONE', *, *, #46304, .F. ) ;
#23343=CARTESIAN_POINT ( 'NONE',  ( 10.39999999999991509, 2.500000000000000000, 0.5928203230275495006 ) ) ;
#23344=VERTEX_POINT ( 'NONE', #93937 ) ;
#23345=ORIENTED_EDGE ( 'NONE', *, *, #2690, .F. ) ;
#23346=AXIS2_PLACEMENT_3D ( 'NONE', #18964, #28160, #128962 ) ;
#23347=EDGE_LOOP ( 'NONE', ( #15918, #42975, #86221, #120946 ) ) ;
#23348=VECTOR ( 'NONE', #46957, 1000.000000000000000 ) ;
#23349=LINE ( 'NONE', #35771, #35954 ) ;
#23350=CIRCLE ( 'NONE', #21306, 0.09999999999999982514 ) ;
#23351=CARTESIAN_POINT ( 'NONE',  ( -9.600000000000006750, 2.500000000000000000, 4.922947341949748257 ) ) ;
#23353=VERTEX_POINT ( 'NONE', #74939 ) ;
#23354=DIRECTION ( 'NONE',  ( -0.000000000000000000, 1.000000000000000000, -0.000000000000000000 ) ) ;
#23355=EDGE_CURVE ( 'NONE', #15344, #60734, #4242, .T. ) ;
#23356=DIRECTION ( 'NONE',  ( -0.000000000000000000, -1.000000000000000000, -0.000000000000000000 ) ) ;
#23357=AXIS2_PLACEMENT_3D ( 'NONE', #79189, #60197, #99471 ) ;
#23358=CIRCLE ( 'NONE', #12885, 0.1000000000000002554 ) ;
#23359=DIRECTION ( 'NONE',  ( 0.000000000000000000, 0.000000000000000000, 1.000000000000000000 ) ) ;
#23361=ORIENTED_EDGE ( 'NONE', *, *, #19073, .T. ) ;
#23362=CONICAL_SURFACE ( 'NONE', #100726, 0.1000000000000000472, 0.003490658503988666988 ) ;
#23363=AXIS2_PLACEMENT_3D ( 'NONE', #53258, #93188, #3510 ) ;
#23364=ADVANCED_FACE ( 'NONE', ( #86021 ), #55935, .T. ) ;
#23365=DIRECTION ( 'NONE',  ( 0.000000000000000000, 0.000000000000000000, 1.000000000000000000 ) ) ;
#23366=EDGE_CURVE ( 'NONE', #70798, #126487, #24006, .T. ) ;
#23367=EDGE_LOOP ( 'NONE', ( #97280, #15394 ) ) ;
#23368=PLANE ( 'NONE',  #72243 ) ;
#23369=AXIS2_PLACEMENT_3D ( 'NONE', #46207, #45578, #5621 ) ;
#23370=ORIENTED_EDGE ( 'NONE', *, *, #70830, .F. ) ;
#23371=ORIENTED_EDGE ( 'NONE', *, *, #89317, .T. ) ;
#23372=DIRECTION ( 'NONE',  ( 0.000000000000000000, -0.9999939076577903929, 0.003490651415223739937 ) ) ;
#23373=CARTESIAN_POINT ( 'NONE',  ( -7.100000000000017408, 12.50000000000000000, -5.022947341949754119 ) ) ;
#23374=ADVANCED_FACE ( 'NONE', ( #66398 ), #99231, .T. ) ;
#23375=EDGE_CURVE ( 'NONE', #55123, #89861, #6806, .T. ) ;
#23376=FACE_OUTER_BOUND ( 'NONE', #126189, .T. ) ;
#23377=EDGE_CURVE ( 'NONE', #38438, #48905, #32356, .T. ) ;
#23378=CARTESIAN_POINT ( 'NONE',  ( 1.649999999999951505, 12.50000000000000000, 2.857883832488649301 ) ) ;
#23379=EDGE_CURVE ( 'NONE', #128651, #86983, #124360, .T. ) ;
#23380=CARTESIAN_POINT ( 'NONE',  ( 9.399999999999915090, 2.500000000000000000, -3.983716857408426293 ) ) ;
#23381=EDGE_LOOP ( 'NONE', ( #57032, #88761 ) ) ;
#23382=ORIENTED_EDGE ( 'NONE', *, *, #115865, .F. ) ;
#23383=DIRECTION ( 'NONE',  ( 0.000000000000000000, -0.9999939076577903929, 0.003490651415223739937 ) ) ;
#23384=DIRECTION ( 'NONE',  ( 0.000000000000000000, 1.000000000000000000, 0.000000000000000000 ) ) ;
#23385=CARTESIAN_POINT ( 'NONE',  ( -3.350000000000028511, 2.500000000000000000, 2.757883832488649656 ) ) ;
#23386=ORIENTED_EDGE ( 'NONE', *, *, #101180, .F. ) ;
#23387=ORIENTED_EDGE ( 'NONE', *, *, #19703, .F. ) ;
#23388=EDGE_CURVE ( 'NONE', #30668, #76885, #46784, .T. ) ;
#23389=CARTESIAN_POINT ( 'NONE',  ( -2.950000000000029932, 12.50000000000000000, -2.165063509461101710 ) ) ;
#23390=VECTOR ( 'NONE', #125504, 1000.000000000000000 ) ;
#23391=EDGE_LOOP ( 'NONE', ( #65181, #54268 ) ) ;
#23392=DIRECTION ( 'NONE',  ( -0.000000000000000000, -1.000000000000000000, -0.000000000000000000 ) ) ;
#23393=DIRECTION ( 'NONE',  ( 0.000000000000000000, 0.000000000000000000, 1.000000000000000000 ) ) ;
#23394=CIRCLE ( 'NONE', #398, 0.09999999999999982514 ) ;
#23395=CARTESIAN_POINT ( 'NONE',  ( -6.650000000000014566, 12.50000000000000000, 1.537336459617582918 ) ) ;
#23396=ORIENTED_EDGE ( 'NONE', *, *, #100691, .F. ) ;
#23397=CARTESIAN_POINT ( 'NONE',  ( 12.04999999999990479, 2.500000000000000000, -6.595190528383302109 ) ) ;
#23398=DIRECTION ( 'NONE',  ( 0.000000000000000000, 0.000000000000000000, -1.000000000000000000 ) ) ;
#23399=DIRECTION ( 'NONE',  ( 0.000000000000000000, 1.000000000000000000, 0.000000000000000000 ) ) ;
#23400=CARTESIAN_POINT ( 'NONE',  ( 12.29999999999990656, 12.50000000000000000, -4.611443907251939756 ) ) ;
#23401=DIRECTION ( 'NONE',  ( -0.000000000000000000, 1.000000000000000000, -0.000000000000000000 ) ) ;
#23402=EDGE_LOOP ( 'NONE', ( #83292, #114661, #61802, #110059 ) ) ;
#23403=VECTOR ( 'NONE', #109701, 1000.000000000000000 ) ;
#23404=AXIS2_PLACEMENT_3D ( 'NONE', #46611, #126474, #27598 ) ;
#23405=DIRECTION ( 'NONE',  ( -4.274815082592931898E-19, -0.9999939076577903929, -0.003490651415223739937 ) ) ;
#23406=AXIS2_PLACEMENT_3D ( 'NONE', #116655, #103134, #82865 ) ;
#23407=CARTESIAN_POINT ( 'NONE',  ( 2.899999999999946620, 2.500000000000000000, -5.022947341949754119 ) ) ;
#23408=ORIENTED_EDGE ( 'NONE', *, *, #65533, .F. ) ;
#23409=( BOUNDED_SURFACE ( )  B_SPLINE_SURFACE ( 3, 2, ( 
 ( #5069, #120508, #30853 ),
 ( #37762, #67184, #86193 ),
 ( #96659, #58061, #76406 ),
 ( #97328, #108427, #106502 ) ),
 .UNSPECIFIED., .F., .F., .F. ) 
 B_SPLINE_SURFACE_WITH_KNOTS ( ( 4, 4 ),
 ( 3, 3 ),
 ( 0.000000000000000000, 0.002140783231465596091 ),
 ( 0.000000000000000000, 1.000000000000000000 ),
 .UNSPECIFIED. ) 
 GEOMETRIC_REPRESENTATION_ITEM ( )  RATIONAL_B_SPLINE_SURFACE ( (
 ( 1.000000000000000000, 0.7071067811865471286, 1.000000000000000000),
 ( 1.000000000000000000, 0.7083221553718337393, 1.000000000000000000),
 ( 1.000000000000000000, 0.7095583407460066550, 1.000000000000000000),
 ( 1.000000000000000000, 0.7108129114090289136, 1.000000000000000000) ) ) 
 REPRESENTATION_ITEM ( '' )  SURFACE ( )  );
#23410=ORIENTED_EDGE ( 'NONE', *, *, #30634, .F. ) ;
#23411=ADVANCED_FACE ( 'NONE', ( #98424 ), #59843, .T. ) ;
#23413=CARTESIAN_POINT ( 'NONE',  ( 6.899999999999928413, 12.50000000000000000, 3.983716857408420964 ) ) ;
#23414=DIRECTION ( 'NONE',  ( 0.000000000000000000, 1.000000000000000000, 0.000000000000000000 ) ) ;
#23415=CONICAL_SURFACE ( 'NONE', #127974, 0.1000000000000002554, 0.003490658503988666988 ) ;
#23416=DIRECTION ( 'NONE',  ( 0.000000000000000000, -0.000000000000000000, 1.000000000000000000 ) ) ;
#23417=CARTESIAN_POINT ( 'NONE',  ( 2.049999999999950084, 12.50000000000000000, 2.099970236277060032 ) ) ;
#23419=CARTESIAN_POINT ( 'NONE',  ( -5.650000000000019895, 2.500000000000000000, 6.841600689897072485 ) ) ;
#23420=CARTESIAN_POINT ( 'NONE',  ( 1.899999999999951283, 12.50000000000000000, -0.3464101615137782364 ) ) ;
#23421=DIRECTION ( 'NONE',  ( 0.000000000000000000, 1.000000000000000000, 0.000000000000000000 ) ) ;
#23422=CIRCLE ( 'NONE', #113306, 0.1000000000000000472 ) ;
#23424=AXIS2_PLACEMENT_3D ( 'NONE', #87760, #47867, #90329 ) ;
#23425=PLANE ( 'NONE',  #4462 ) ;
#23426=EDGE_CURVE ( 'NONE', #80635, #96252, #39560, .T. ) ;
#23427=EDGE_CURVE ( 'NONE', #25583, #114104, #107630, .T. ) ;
#23429=ADVANCED_FACE ( 'NONE', ( #109559 ), #65759, .T. ) ;
#23430=DIRECTION ( 'NONE',  ( 0.000000000000000000, 1.000000000000000000, 0.000000000000000000 ) ) ;
#23431=VERTEX_POINT ( 'NONE', #68335 ) ;
#23432=ORIENTED_EDGE ( 'NONE', *, *, #114616, .F. ) ;
#23433=ADVANCED_FACE ( 'NONE', ( #88624 ), #10066, .T. ) ;
#23434=AXIS2_PLACEMENT_3D ( 'NONE', #128996, #68099, #9833 ) ;
#23435=ORIENTED_EDGE ( 'NONE', *, *, #99087, .T. ) ;
#23436=ADVANCED_FACE ( 'NONE', ( #58538 ), #115944, .T. ) ;
#23437=ORIENTED_EDGE ( 'NONE', *, *, #64224, .T. ) ;
#23438=ADVANCED_FACE ( 'NONE', ( #128581 ), #34487, .T. ) ;
#23439=FACE_OUTER_BOUND ( 'NONE', #98727, .T. ) ;
#23440=DIRECTION ( 'NONE',  ( 0.000000000000000000, -0.9999939076577903929, 0.003490651415223739937 ) ) ;
#23441=EDGE_CURVE ( 'NONE', #49455, #98528, #82512, .T. ) ;
#23442=ORIENTED_EDGE ( 'NONE', *, *, #124974, .T. ) ;
#23443=EDGE_CURVE ( 'NONE', #72025, #92653, #109694, .T. ) ;
#23444=DIRECTION ( 'NONE',  ( 0.000000000000000000, 0.000000000000000000, 1.000000000000000000 ) ) ;
#23445=EDGE_CURVE ( 'NONE', #119499, #75029, #29706, .T. ) ;
#23446=CARTESIAN_POINT ( 'NONE',  ( -5.000000000000023093, 2.500000000000000000, 0.6928203230275494784 ) ) ;
#23448=ORIENTED_EDGE ( 'NONE', *, *, #69788, .T. ) ;
#23449=DIRECTION ( 'NONE',  ( 0.000000000000000000, 0.000000000000000000, -1.000000000000000000 ) ) ;
#23450=ADVANCED_FACE ( 'NONE', ( #106959 ), #7474, .T. ) ;
#23451=DIRECTION ( 'NONE',  ( -0.000000000000000000, -1.000000000000000000, -0.000000000000000000 ) ) ;
#23452=VERTEX_POINT ( 'NONE', #127272 ) ;
#23453=ORIENTED_EDGE ( 'NONE', *, *, #30215, .F. ) ;
#23454=ORIENTED_EDGE ( 'NONE', *, *, #13602, .T. ) ;
#23455=CIRCLE ( 'NONE', #128011, 0.09999999999999999167 ) ;
#23456=EDGE_LOOP ( 'NONE', ( #113429, #28230, #86482, #24508 ) ) ;
#23457=DIRECTION ( 'NONE',  ( 0.000000000000000000, 0.000000000000000000, 1.000000000000000000 ) ) ;
#23458=AXIS2_PLACEMENT_3D ( 'NONE', #95116, #27020, #117959 ) ;
#23459=AXIS2_PLACEMENT_3D ( 'NONE', #109382, #19728, #60313 ) ;
#23460=CARTESIAN_POINT ( 'NONE',  ( -5.400000000000023448, 12.50000000000000000, -4.330127018922201643 ) ) ;
#23461=CARTESIAN_POINT ( 'NONE',  ( -4.400000000000025224, 2.500000000000000000, 4.576537180435972019 ) ) ;
#23462=LINE ( 'NONE', #32675, #62468 ) ;
#23463=AXIS2_PLACEMENT_3D ( 'NONE', #105903, #46329, #19442 ) ;
#23464=ORIENTED_EDGE ( 'NONE', *, *, #44603, .F. ) ;
#23465=AXIS2_PLACEMENT_3D ( 'NONE', #53702, #34736, #22964 ) ;
#23466=AXIS2_PLACEMENT_3D ( 'NONE', #55824, #5423, #45377 ) ;
#23467=LINE ( 'NONE', #24767, #127604 ) ;
#23468=CIRCLE ( 'NONE', #117531, 0.09999999999999982514 ) ;
#23469=ORIENTED_EDGE ( 'NONE', *, *, #56624, .F. ) ;
#23470=CARTESIAN_POINT ( 'NONE',  ( 1.849999999999949019, 2.500000000000000000, 6.741600689897071952 ) ) ;
#23471=CARTESIAN_POINT ( 'NONE',  ( -0.4000000000000331624, 2.500000000000000000, -0.6928203230275519209 ) ) ;
#23472=AXIS2_PLACEMENT_3D ( 'NONE', #96793, #65406, #86330 ) ;
#23473=CARTESIAN_POINT ( 'NONE',  ( -10.40000000000000213, 2.500000000000000000, 5.022947341949748790 ) ) ;
#23474=CARTESIAN_POINT ( 'NONE',  ( 10.19999999999991225, 2.500000000000000000, 3.983716857408420076 ) ) ;
#23475=AXIS2_PLACEMENT_3D ( 'NONE', #91530, #73177, #81697 ) ;
#23476=ORIENTED_EDGE ( 'NONE', *, *, #32708, .T. ) ;
#23477=ORIENTED_EDGE ( 'NONE', *, *, #43555, .T. ) ;
#23478=ORIENTED_EDGE ( 'NONE', *, *, #34, .T. ) ;
#23479=CARTESIAN_POINT ( 'NONE',  ( 0.8499999999999553468, 12.50000000000000000, -2.857883832488653741 ) ) ;
#23480=DIRECTION ( 'NONE',  ( -0.000000000000000000, 1.000000000000000000, -0.000000000000000000 ) ) ;
#23481=FACE_OUTER_BOUND ( 'NONE', #104236, .T. ) ;
#23482=FACE_BOUND ( 'NONE', #47507, .T. ) ;
#23483=PLANE ( 'NONE',  #45097 ) ;
#23484=CARTESIAN_POINT ( 'NONE',  ( -2.050000000000033129, 2.500000000000000000, 6.395190528383296602 ) ) ;
#23485=CARTESIAN_POINT ( 'NONE',  ( 13.14999999999989733, 2.500000000000000000, -1.918653347947325782 ) ) ;
#23486=ADVANCED_FACE ( 'NONE', ( #57227 ), #83817, .T. ) ;
#23487=DIRECTION ( 'NONE',  ( 0.000000000000000000, 0.000000000000000000, 1.000000000000000000 ) ) ;
#23488=CARTESIAN_POINT ( 'NONE',  ( 7.099999999999925926, 2.500000000000000000, 0.7928203230275495672 ) ) ;
#23489=DIRECTION ( 'NONE',  ( 0.000000000000000000, -0.9999939076577903929, 0.003490651415223739937 ) ) ;
#23490=ORIENTED_EDGE ( 'NONE', *, *, #15292, .F. ) ;
#23491=AXIS2_PLACEMENT_3D ( 'NONE', #110229, #112167, #24425 ) ;
#23492=DIRECTION ( 'NONE',  ( -0.000000000000000000, -1.000000000000000000, -0.000000000000000000 ) ) ;
#23493=ORIENTED_EDGE ( 'NONE', *, *, #123129, .T. ) ;
#23494=VERTEX_POINT ( 'NONE', #108889 ) ;
#23495=EDGE_CURVE ( 'NONE', #949, #4124, #81674, .T. ) ;
#23496=CARTESIAN_POINT ( 'NONE',  ( -6.050000000000020250, 12.50000000000000000, -6.841600689897078702 ) ) ;
#23497=FACE_BOUND ( 'NONE', #93532, .T. ) ;
#23498=VECTOR ( 'NONE', #18644, 1000.000000000000000 ) ;
#23499=DIRECTION ( 'NONE',  ( -0.000000000000000000, 1.000000000000000000, -0.000000000000000000 ) ) ;
#23500=AXIS2_PLACEMENT_3D ( 'NONE', #62975, #14500, #112085 ) ;
#23501=CIRCLE ( 'NONE', #107117, 0.06509327318403745899 ) ;
#23502=ORIENTED_EDGE ( 'NONE', *, *, #119914, .F. ) ;
#23503=CARTESIAN_POINT ( 'NONE',  ( 32.15727368888380511, 2.842525632570505500, 4.549395963655256558 ) ) ;
#23504=DIRECTION ( 'NONE',  ( 0.000000000000000000, 0.000000000000000000, -1.000000000000000000 ) ) ;
#23505=ORIENTED_EDGE ( 'NONE', *, *, #103490, .F. ) ;
#23506=AXIS2_PLACEMENT_3D ( 'NONE', #1270, #41219, #89013 ) ;
#23507=DIRECTION ( 'NONE',  ( -0.000000000000000000, -1.000000000000000000, -0.000000000000000000 ) ) ;
#23509=CIRCLE ( 'NONE', #128080, 0.1000000000000000472 ) ;
#23510=CIRCLE ( 'NONE', #36046, 0.09999999999999999167 ) ;
#23511=AXIS2_PLACEMENT_3D ( 'NONE', #109376, #40008, #50451 ) ;
#23512=CIRCLE ( 'NONE', #52760, 0.1000000000000002554 ) ;
#23513=EDGE_LOOP ( 'NONE', ( #50334, #96768, #73208, #68702 ) ) ;
#23514=CARTESIAN_POINT ( 'NONE',  ( -5.650000000000023448, 12.50000000000000000, -6.841600689897078702 ) ) ;
#23515=DIRECTION ( 'NONE',  ( 0.000000000000000000, -0.9999939076577903929, 0.003490651415223739937 ) ) ;
#23516=AXIS2_PLACEMENT_3D ( 'NONE', #107213, #66002, #105932 ) ;
#23517=VERTEX_POINT ( 'NONE', #78171 ) ;
#23518=EDGE_CURVE ( 'NONE', #128651, #124598, #59180, .T. ) ;
#23519=DIRECTION ( 'NONE',  ( -4.274815082592931898E-19, -0.9999939076577903929, -0.003490651415223739937 ) ) ;
#23520=CIRCLE ( 'NONE', #88259, 0.1000000000000002554 ) ;
#23522=CARTESIAN_POINT ( 'NONE',  ( -9.350000000000006750, 12.50000000000000000, -1.883746621131363375 ) ) ;
#23523=EDGE_LOOP ( 'NONE', ( #52518, #118582 ) ) ;
#23524=ORIENTED_EDGE ( 'NONE', *, *, #116275, .T. ) ;
#23525=CARTESIAN_POINT ( 'NONE',  ( -11.64999999999999858, 2.500000000000000000, -1.372243186433546036 ) ) ;
#23526=EDGE_CURVE ( 'NONE', #26624, #45516, #101019, .T. ) ;
#23527=ORIENTED_EDGE ( 'NONE', *, *, #32590, .T. ) ;
#23528=DIRECTION ( 'NONE',  ( 0.000000000000000000, 0.000000000000000000, 1.000000000000000000 ) ) ;
#23529=FACE_OUTER_BOUND ( 'NONE', #34211, .T. ) ;
#23530=EDGE_LOOP ( 'NONE', ( #12873, #46701, #60165, #53480 ) ) ;
#23531=CARTESIAN_POINT ( 'NONE',  ( 2.299999999999946976, 2.500000000000000000, 4.576537180435972019 ) ) ;
#23532=CARTESIAN_POINT ( 'NONE',  ( 11.24999999999994316, 12.50000000000000000, 2.165063509461097713 ) ) ;
#23533=DIRECTION ( 'NONE',  ( 0.000000000000000000, 0.000000000000000000, 1.000000000000000000 ) ) ;
#23534=ADVANCED_FACE ( 'NONE', ( #62400 ), #64940, .T. ) ;
#23535=EDGE_CURVE ( 'NONE', #7221, #85421, #120667, .T. ) ;
#23536=DIRECTION ( 'NONE',  ( 0.000000000000000000, 1.000000000000000000, 0.000000000000000000 ) ) ;
#23537=CIRCLE ( 'NONE', #29811, 0.06509327318403745899 ) ;
#23538=EDGE_CURVE ( 'NONE', #31627, #41779, #42108, .T. ) ;
#23539=ADVANCED_FACE ( 'NONE', ( #101676 ), #21165, .T. ) ;
#23540=EDGE_CURVE ( 'NONE', #109349, #11815, #100545, .T. ) ;
#23541=FACE_OUTER_BOUND ( 'NONE', #1777, .T. ) ;
#23542=VERTEX_POINT ( 'NONE', #52561 ) ;
#23543=ORIENTED_EDGE ( 'NONE', *, *, #39690, .F. ) ;
#23544=CARTESIAN_POINT ( 'NONE',  ( -6.850000000000013856, 2.500000000000000000, 1.818653347947321475 ) ) ;
#23545=AXIS2_PLACEMENT_3D ( 'NONE', #91927, #54557, #84022 ) ;
#23548=AXIS2_PLACEMENT_3D ( 'NONE', #50800, #93299, #111654 ) ;
#23549=ORIENTED_EDGE ( 'NONE', *, *, #105961, .T. ) ;
#23550=ORIENTED_EDGE ( 'NONE', *, *, #103067, .T. ) ;
#23551=ORIENTED_EDGE ( 'NONE', *, *, #77075, .T. ) ;
#23552=ADVANCED_FACE ( 'NONE', ( #112140 ), #25220, .T. ) ;
#23553=CARTESIAN_POINT ( 'NONE',  ( 1.249999999999988454, 12.50000000000000000, -2.165063509461101710 ) ) ;
#23554=ADVANCED_FACE ( 'NONE', ( #32952 ), #39924, .T. ) ;
#23556=VECTOR ( 'NONE', #11171, 1000.000000000000000 ) ;
#23557=ADVANCED_FACE ( 'NONE', ( #22488 ), #127641, .T. ) ;
#23558=CIRCLE ( 'NONE', #96700, 0.06509327318403745899 ) ;
#23559=CARTESIAN_POINT ( 'NONE',  ( 10.59999999999991260, 2.500000000000000000, -0.4464101615137783252 ) ) ;
#23560=AXIS2_PLACEMENT_3D ( 'NONE', #22014, #61932, #3003 ) ;
#23561=CARTESIAN_POINT ( 'NONE',  ( -0.4000000000000401013, 2.500000000000000000, -3.737306695894649700 ) ) ;
#23562=DIRECTION ( 'NONE',  ( -0.000000000000000000, 1.000000000000000000, -0.000000000000000000 ) ) ;
#23563=CARTESIAN_POINT ( 'NONE',  ( 4.799999999999937650, 2.500000000000000000, -0.3464101615137782364 ) ) ;
#23564=AXIS2_PLACEMENT_3D ( 'NONE', #10027, #40131, #1482 ) ;
#23565=DIRECTION ( 'NONE',  ( -0.000000000000000000, 1.000000000000000000, -0.000000000000000000 ) ) ;
#23566=DIRECTION ( 'NONE',  ( 0.000000000000000000, 1.000000000000000000, 0.000000000000000000 ) ) ;
#23567=AXIS2_PLACEMENT_3D ( 'NONE', #39631, #50092, #59912 ) ;
#23568=CONICAL_SURFACE ( 'NONE', #7107, 0.1000000000000002554, 0.003490658503988666988 ) ;
#23570=VERTEX_POINT ( 'NONE', #100382 ) ;
#23571=LINE ( 'NONE', #65423, #111232 ) ;
#23572=VERTEX_POINT ( 'NONE', #60478 ) ;
#23573=ORIENTED_EDGE ( 'NONE', *, *, #76617, .F. ) ;
#23574=FACE_OUTER_BOUND ( 'NONE', #76915, .T. ) ;
#23576=CARTESIAN_POINT ( 'NONE',  ( -5.850000000000018296, 2.500000000000000000, 2.857883832488649301 ) ) ;
#23578=DIRECTION ( 'NONE',  ( 0.000000000000000000, 1.000000000000000000, 0.000000000000000000 ) ) ;
#23580=DIRECTION ( 'NONE',  ( 0.000000000000000000, 0.000000000000000000, 1.000000000000000000 ) ) ;
#23581=EDGE_LOOP ( 'NONE', ( #8847, #481 ) ) ;
#23582=CARTESIAN_POINT ( 'NONE',  ( -3.300000000000028244, 2.500000000000000000, 4.430127018922196847 ) ) ;
#23584=AXIS2_PLACEMENT_3D ( 'NONE', #299, #120106, #118161 ) ;
#23585=ORIENTED_EDGE ( 'NONE', *, *, #32175, .T. ) ;
#23586=CONICAL_SURFACE ( 'NONE', #113470, 0.1000000000000002554, 0.003490658503988666988 ) ;
#23587=ORIENTED_EDGE ( 'NONE', *, *, #77347, .T. ) ;
#23588=VERTEX_POINT ( 'NONE', #50630 ) ;
#23589=EDGE_CURVE ( 'NONE', #114788, #114154, #51301, .T. ) ;
#23590=VERTEX_POINT ( 'NONE', #112783 ) ;
#23591=CONICAL_SURFACE ( 'NONE', #38277, 0.09999999999999982514, 0.003490658503988666988 ) ;
#23592=DIRECTION ( 'NONE',  ( 0.000000000000000000, 0.000000000000000000, 1.000000000000000000 ) ) ;
#23593=CARTESIAN_POINT ( 'NONE',  ( 7.699999999999925571, 2.500000000000000000, 3.983716857408420076 ) ) ;
#23594=VECTOR ( 'NONE', #15836, 1000.000000000000000 ) ;
#23595=ADVANCED_FACE ( 'NONE', ( #43413 ), #119321, .T. ) ;
#23596=CIRCLE ( 'NONE', #57036, 0.06509327318403745899 ) ;
#23597=DIRECTION ( 'NONE',  ( -0.000000000000000000, 1.000000000000000000, -0.000000000000000000 ) ) ;
#23598=CIRCLE ( 'NONE', #44528, 0.1000000000000002554 ) ;
#23599=DIRECTION ( 'NONE',  ( -0.000000000000000000, 1.000000000000000000, -0.000000000000000000 ) ) ;
#23600=ADVANCED_FACE ( 'NONE', ( #10680 ), #41485, .T. ) ;
#23601=DIRECTION ( 'NONE',  ( 0.000000000000000000, -0.9999939076577903929, 0.003490651415223739937 ) ) ;
#23602=VERTEX_POINT ( 'NONE', #102948 ) ;
#23603=DIRECTION ( 'NONE',  ( 0.000000000000000000, 1.000000000000000000, 0.000000000000000000 ) ) ;
#23604=CARTESIAN_POINT ( 'NONE',  ( 8.749999999999957367, 2.500000000000000000, 2.065063509461097624 ) ) ;
#23605=DIRECTION ( 'NONE',  ( -0.000000000000000000, -1.000000000000000000, -0.000000000000000000 ) ) ;
#23606=CIRCLE ( 'NONE', #90397, 0.09999999999999999167 ) ;
#23607=EDGE_CURVE ( 'NONE', #54302, #13172, #48230, .T. ) ;
#23608=CONICAL_SURFACE ( 'NONE', #90398, 0.1000000000000002554, 0.003490658503988666988 ) ;
#23609=CARTESIAN_POINT ( 'NONE',  ( 8.749999999999957367, 2.500000000000000000, -6.495190528383302464 ) ) ;
#23610=ORIENTED_EDGE ( 'NONE', *, *, #69313, .F. ) ;
#23611=AXIS2_PLACEMENT_3D ( 'NONE', #88704, #101101, #59267 ) ;
#23612=AXIS2_PLACEMENT_3D ( 'NONE', #107930, #6469, #77818 ) ;
#23613=CIRCLE ( 'NONE', #38203, 0.09999999999999982514 ) ;
#23614=ORIENTED_EDGE ( 'NONE', *, *, #67559, .T. ) ;
#23615=ORIENTED_EDGE ( 'NONE', *, *, #63499, .F. ) ;
#23616=DIRECTION ( 'NONE',  ( 0.000000000000000000, 0.000000000000000000, 1.000000000000000000 ) ) ;
#23617=AXIS2_PLACEMENT_3D ( 'NONE', #103850, #101266, #3075 ) ;
#23618=DIRECTION ( 'NONE',  ( -0.000000000000000000, -1.000000000000000000, -0.000000000000000000 ) ) ;
#23619=CARTESIAN_POINT ( 'NONE',  ( 13.09999999999989839, 2.500000000000000000, 0.4464101615137735513 ) ) ;
#23620=AXIS2_PLACEMENT_3D ( 'NONE', #90151, #70530, #100623 ) ;
#23621=ORIENTED_EDGE ( 'NONE', *, *, #50028, .T. ) ;
#23622=DIRECTION ( 'NONE',  ( 0.000000000000000000, 0.000000000000000000, 1.000000000000000000 ) ) ;
#23623=FACE_OUTER_BOUND ( 'NONE', #101793, .T. ) ;
#23624=CARTESIAN_POINT ( 'NONE',  ( 11.64999999999990798, 2.500000000000000000, 5.802370205355744659 ) ) ;
#23626=DIRECTION ( 'NONE',  ( 0.000000000000000000, 0.000000000000000000, 1.000000000000000000 ) ) ;
#23627=DIRECTION ( 'NONE',  ( 0.000000000000000000, 0.000000000000000000, 1.000000000000000000 ) ) ;
#23628=VERTEX_POINT ( 'NONE', #76077 ) ;
#23629=CIRCLE ( 'NONE', #128101, 0.09999999999999982514 ) ;
#23630=ORIENTED_EDGE ( 'NONE', *, *, #114163, .T. ) ;
#23631=AXIS2_PLACEMENT_3D ( 'NONE', #51146, #91054, #13116 ) ;
#23632=LINE ( 'NONE', #13147, #43919 ) ;
#23633=DIRECTION ( 'NONE',  ( 0.000000000000000000, 0.000000000000000000, 1.000000000000000000 ) ) ;
#23634=CARTESIAN_POINT ( 'NONE',  ( 4.549999999999939426, 2.500000000000000000, -6.395190528383301931 ) ) ;
#23635=CARTESIAN_POINT ( 'NONE',  ( -5.650000000000019895, 2.500000000000000000, 1.818653347947321475 ) ) ;
#23636=FACE_OUTER_BOUND ( 'NONE', #71058, .T. ) ;
#23637=EDGE_LOOP ( 'NONE', ( #94774, #24639 ) ) ;
#23638=CONICAL_SURFACE ( 'NONE', #36472, 0.1000000000000002554, 0.003490658503988666988 ) ;
#23639=EDGE_CURVE ( 'NONE', #33187, #50793, #6419, .T. ) ;
#23640=AXIS2_PLACEMENT_3D ( 'NONE', #74220, #33652, #112860 ) ;
#23641=VECTOR ( 'NONE', #114493, 1000.000000000000000 ) ;
#23642=VECTOR ( 'NONE', #46786, 1000.000000000000000 ) ;
#23643=ORIENTED_EDGE ( 'NONE', *, *, #47093, .F. ) ;
#23644=FACE_OUTER_BOUND ( 'NONE', #47514, .T. ) ;
#23645=DIRECTION ( 'NONE',  ( 0.000000000000000000, 0.000000000000000000, 1.000000000000000000 ) ) ;
#23646=DIRECTION ( 'NONE',  ( 0.000000000000000000, 1.000000000000000000, 0.000000000000000000 ) ) ;
#23647=CARTESIAN_POINT ( 'NONE',  ( -8.100000000000010303, 12.50000000000000000, 3.983716857408420964 ) ) ;
#23648=ORIENTED_EDGE ( 'NONE', *, *, #11420, .T. ) ;
#23649=AXIS2_PLACEMENT_3D ( 'NONE', #97663, #9288, #68194 ) ;
#23650=CARTESIAN_POINT ( 'NONE',  ( -6.050000000000020250, 12.50000000000000000, -2.511473670974877948 ) ) ;
#23651=CIRCLE ( 'NONE', #15217, 0.06509327318403745899 ) ;
#23652=VECTOR ( 'NONE', #101693, 1000.000000000000000 ) ;
#23653=DIRECTION ( 'NONE',  ( -0.000000000000000000, -1.000000000000000000, -0.000000000000000000 ) ) ;
#23654=CIRCLE ( 'NONE', #119795, 0.06509327318403745899 ) ;
#23655=ORIENTED_EDGE ( 'NONE', *, *, #4301, .F. ) ;
#23656=CIRCLE ( 'NONE', #69723, 0.1000000000000000472 ) ;
#23657=DIRECTION ( 'NONE',  ( 0.000000000000000000, 0.000000000000000000, 1.000000000000000000 ) ) ;
#23658=EDGE_CURVE ( 'NONE', #37153, #72458, #94279, .T. ) ;
#23659=ORIENTED_EDGE ( 'NONE', *, *, #19271, .T. ) ;
#23660=CONICAL_SURFACE ( 'NONE', #25713, 0.1000000000000002554, 0.003490658503988666988 ) ;
#23661=CARTESIAN_POINT ( 'NONE',  ( 0.8499999999999553468, 2.500000000000000000, -2.857883832488653741 ) ) ;
#23662=ORIENTED_EDGE ( 'NONE', *, *, #11996, .F. ) ;
#23663=CARTESIAN_POINT ( 'NONE',  ( 1.249999999999952038, 2.500000000000000000, 5.802370205355744659 ) ) ;
#23664=CARTESIAN_POINT ( 'NONE',  ( -5.650000000000019895, 12.50000000000000000, 6.148780366869520009 ) ) ;
#23665=EDGE_LOOP ( 'NONE', ( #111851, #108256 ) ) ;
#23666=ORIENTED_EDGE ( 'NONE', *, *, #92992, .T. ) ;
#23668=CARTESIAN_POINT ( 'NONE',  ( -13.09999999999999254, 2.500000000000000000, -3.983716857408423628 ) ) ;
#23669=CONICAL_SURFACE ( 'NONE', #36206, 0.1000000000000000472, 0.003490658503988666988 ) ;
#23672=DIRECTION ( 'NONE',  ( -0.000000000000000000, 1.000000000000000000, -0.000000000000000000 ) ) ;
#23673=DIRECTION ( 'NONE',  ( 0.000000000000000000, 0.000000000000000000, -1.000000000000000000 ) ) ;
#23674=DIRECTION ( 'NONE',  ( 0.000000000000000000, 0.000000000000000000, -1.000000000000000000 ) ) ;
#23675=LINE ( 'NONE', #92408, #42132 ) ;
#23676=AXIS2_PLACEMENT_3D ( 'NONE', #124889, #75145, #65302 ) ;
#23677=AXIS2_PLACEMENT_3D ( 'NONE', #46695, #73557, #14628 ) ;
#23678=ORIENTED_EDGE ( 'NONE', *, *, #78567, .T. ) ;
#23679=ADVANCED_FACE ( 'NONE', ( #56421 ), #125572, .T. ) ;
#23680=ORIENTED_EDGE ( 'NONE', *, *, #69786, .F. ) ;
#23681=DIRECTION ( 'NONE',  ( -0.000000000000000000, 1.000000000000000000, -0.000000000000000000 ) ) ;
#23682=ORIENTED_EDGE ( 'NONE', *, *, #120243, .F. ) ;
#23683=DIRECTION ( 'NONE',  ( 0.000000000000000000, 0.000000000000000000, 1.000000000000000000 ) ) ;
#23684=DIRECTION ( 'NONE',  ( 0.000000000000000000, 1.000000000000000000, 0.000000000000000000 ) ) ;
#23685=DIRECTION ( 'NONE',  ( -0.000000000000000000, -1.000000000000000000, -0.000000000000000000 ) ) ;
#23686=ORIENTED_EDGE ( 'NONE', *, *, #58152, .T. ) ;
#23687=ORIENTED_EDGE ( 'NONE', *, *, #3504, .F. ) ;
#23688=CARTESIAN_POINT ( 'NONE',  ( 0.000000000000000000, 2.500000000000000000, 0.000000000000000000 ) ) ;
#23689=ORIENTED_EDGE ( 'NONE', *, *, #10255, .F. ) ;
#23690=EDGE_CURVE ( 'NONE', #76936, #30682, #63686, .T. ) ;
#23691=CIRCLE ( 'NONE', #122086, 0.1000000000000002554 ) ;
#23692=FACE_OUTER_BOUND ( 'NONE', #99651, .T. ) ;
#23694=AXIS2_PLACEMENT_3D ( 'NONE', #56088, #86842, #16788 ) ;
#23695=AXIS2_PLACEMENT_3D ( 'NONE', #65877, #1950, #122395 ) ;
#23696=DIRECTION ( 'NONE',  ( 0.000000000000000000, -0.9999939076577903929, 0.003490651415223739937 ) ) ;
#23697=EDGE_CURVE ( 'NONE', #1010, #104091, #79623, .T. ) ;
#23698=DIRECTION ( 'NONE',  ( -4.274815082592931898E-19, -0.9999939076577903929, -0.003490651415223739937 ) ) ;
#23699=CARTESIAN_POINT ( 'NONE',  ( 0.8499999999999545697, 2.500000000000000000, -1.572243186433550211 ) ) ;
#23700=CARTESIAN_POINT ( 'NONE',  ( -0.8500000000000382805, 12.50000000000000000, -7.122917578226816815 ) ) ;
#23701=CARTESIAN_POINT ( 'NONE',  ( 2.899999999999946620, 2.500000000000000000, -3.637306695894650055 ) ) ;
#23702=CARTESIAN_POINT ( 'NONE',  ( 9.999999999999952038, 2.500000000000000000, -2.276824562219559311E-15 ) ) ;
#23703=EDGE_CURVE ( 'NONE', #117167, #12607, #92131, .T. ) ;
#23704=EDGE_CURVE ( 'NONE', #18200, #55354, #60841, .T. ) ;
#23705=DIRECTION ( 'NONE',  ( -0.000000000000000000, -1.000000000000000000, -0.000000000000000000 ) ) ;
#23706=CARTESIAN_POINT ( 'NONE',  ( -1.650000000000034328, 12.50000000000000000, -2.792790559304616504 ) ) ;
#23707=EDGE_CURVE ( 'NONE', #99701, #103573, #113062, .T. ) ;
#23708=EDGE_CURVE ( 'NONE', #107893, #23087, #56609, .T. ) ;
#23709=FACE_OUTER_BOUND ( 'NONE', #112006, .T. ) ;
#23710=ORIENTED_EDGE ( 'NONE', *, *, #74240, .F. ) ;
#23711=EDGE_LOOP ( 'NONE', ( #54915, #51897 ) ) ;
#23712=ORIENTED_EDGE ( 'NONE', *, *, #54768, .T. ) ;
#23713=FACE_OUTER_BOUND ( 'NONE', #118735, .T. ) ;
#23714=VECTOR ( 'NONE', #80154, 1000.000000000000000 ) ;
#23715=ORIENTED_EDGE ( 'NONE', *, *, #110048, .F. ) ;
#23716=AXIS2_PLACEMENT_3D ( 'NONE', #107900, #98711, #77158 ) ;
#23717=ADVANCED_FACE ( 'NONE', ( #104868 ), #65603, .T. ) ;
#23718=CARTESIAN_POINT ( 'NONE',  ( -6.850000000000017408, 2.500000000000000000, -6.048780366869526581 ) ) ;
#23719=EDGE_CURVE ( 'NONE', #25933, #77313, #2238, .T. ) ;
#23720=ORIENTED_EDGE ( 'NONE', *, *, #56536, .T. ) ;
#23721=ORIENTED_EDGE ( 'NONE', *, *, #102567, .F. ) ;
#23722=EDGE_LOOP ( 'NONE', ( #101682, #99818 ) ) ;
#23723=CIRCLE ( 'NONE', #55113, 0.06509327318403745899 ) ;
#23724=EDGE_CURVE ( 'NONE', #93103, #80552, #73351, .T. ) ;
#23727=EDGE_CURVE ( 'NONE', #16935, #82756, #67064, .T. ) ;
#23728=LINE ( 'NONE', #24366, #101206 ) ;
#23729=DIRECTION ( 'NONE',  ( 0.000000000000000000, 1.000000000000000000, 0.000000000000000000 ) ) ;
#23730=DIRECTION ( 'NONE',  ( -0.000000000000000000, 1.000000000000000000, -0.000000000000000000 ) ) ;
#23731=CARTESIAN_POINT ( 'NONE',  ( 12.29999999999990123, 12.50000000000000000, 0.4115034346978109769 ) ) ;
#23732=CARTESIAN_POINT ( 'NONE',  ( 7.299999999999926104, 2.500000000000000000, -0.2464101615137782308 ) ) ;
#23733=ORIENTED_EDGE ( 'NONE', *, *, #120506, .T. ) ;
#23734=ADVANCED_FACE ( 'NONE', ( #44687 ), #106798, .T. ) ;
#23735=CARTESIAN_POINT ( 'NONE',  ( 12.49999999999990585, 2.500000000000000000, -5.122947341949753763 ) ) ;
#23736=ORIENTED_EDGE ( 'NONE', *, *, #126407, .F. ) ;
#23737=ORIENTED_EDGE ( 'NONE', *, *, #116754, .F. ) ;
#23738=ORIENTED_EDGE ( 'NONE', *, *, #112201, .F. ) ;
#23739=CARTESIAN_POINT ( 'NONE',  ( -4.350000000000023626, 2.500000000000000000, 2.611473670974873151 ) ) ;
#23740=AXIS2_PLACEMENT_3D ( 'NONE', #66704, #45158, #86339 ) ;
#23741=CONICAL_SURFACE ( 'NONE', #44567, 0.1000000000000002554, 0.003490658503988666988 ) ;
#23742=ORIENTED_EDGE ( 'NONE', *, *, #101030, .T. ) ;
#23743=VERTEX_POINT ( 'NONE', #124538 ) ;
#23744=VERTEX_POINT ( 'NONE', #34884 ) ;
#23745=DIRECTION ( 'NONE',  ( -0.000000000000000000, 1.000000000000000000, -0.000000000000000000 ) ) ;
#23746=CIRCLE ( 'NONE', #34115, 0.06509327318403745899 ) ;
#23747=CARTESIAN_POINT ( 'NONE',  ( 3.149999999999946176, 12.50000000000000000, -1.818653347947325916 ) ) ;
#23748=CIRCLE ( 'NONE', #44673, 0.1000000000000002554 ) ;
#23749=CARTESIAN_POINT ( 'NONE',  ( 9.999999999999952038, 2.500000000000000000, -2.276824562219559311E-15 ) ) ;
#23750=CIRCLE ( 'NONE', #32167, 0.06509327318403745899 ) ;
#23751=DIRECTION ( 'NONE',  ( -0.000000000000000000, -1.000000000000000000, -0.000000000000000000 ) ) ;
#23752=DIRECTION ( 'NONE',  ( -0.000000000000000000, -1.000000000000000000, -0.000000000000000000 ) ) ;
#23753=AXIS2_PLACEMENT_3D ( 'NONE', #14195, #46244, #16118 ) ;
#23754=CIRCLE ( 'NONE', #42540, 0.06509327318403745899 ) ;
#23755=DIRECTION ( 'NONE',  ( 0.000000000000000000, 0.000000000000000000, 1.000000000000000000 ) ) ;
#23756=LINE ( 'NONE', #44681, #38805 ) ;
#23757=CIRCLE ( 'NONE', #113629, 0.09999999999999982514 ) ;
#23758=ORIENTED_EDGE ( 'NONE', *, *, #91626, .F. ) ;
#23759=CARTESIAN_POINT ( 'NONE',  ( 11.44999999999990870, 2.500000000000000000, 6.941600689897073018 ) ) ;
#23760=AXIS2_PLACEMENT_3D ( 'NONE', #8666, #119941, #128494 ) ;
#23761=ORIENTED_EDGE ( 'NONE', *, *, #120335, .T. ) ;
#23762=CARTESIAN_POINT ( 'NONE',  ( 7.299999999999926104, 12.50000000000000000, 4.676537180435972552 ) ) ;
#23763=AXIS2_PLACEMENT_3D ( 'NONE', #116271, #14197, #63965 ) ;
#23764=ORIENTED_EDGE ( 'NONE', *, *, #12608, .T. ) ;
#23765=ORIENTED_EDGE ( 'NONE', *, *, #102720, .F. ) ;
#23766=CARTESIAN_POINT ( 'NONE',  ( -5.850000000000021849, 12.50000000000000000, -7.188010851410854052 ) ) ;
#23767=LINE ( 'NONE', #71561, #100759 ) ;
#23768=EDGE_CURVE ( 'NONE', #107010, #3741, #33655, .T. ) ;
#23769=DIRECTION ( 'NONE',  ( -0.000000000000000000, 1.000000000000000000, -0.000000000000000000 ) ) ;
#23770=EDGE_CURVE ( 'NONE', #39659, #107424, #10636, .T. ) ;
#23771=VERTEX_POINT ( 'NONE', #77366 ) ;
#23772=EDGE_LOOP ( 'NONE', ( #127601, #46441 ) ) ;
#23773=DIRECTION ( 'NONE',  ( 0.000000000000000000, 0.000000000000000000, 1.000000000000000000 ) ) ;
#23774=CARTESIAN_POINT ( 'NONE',  ( 10.84999999999991260, 2.500000000000000000, 7.188010851410848723 ) ) ;
#23775=DIRECTION ( 'NONE',  ( 0.000000000000000000, 0.000000000000000000, 1.000000000000000000 ) ) ;
#23776=CARTESIAN_POINT ( 'NONE',  ( -6.650000000000019007, 2.500000000000000000, -5.702370205355749455 ) ) ;
#23777=CONICAL_SURFACE ( 'NONE', #122068, 0.09999999999999982514, 0.003490658503988666988 ) ;
#23778=EDGE_CURVE ( 'NONE', #129312, #128693, #57733, .T. ) ;
#23779=CARTESIAN_POINT ( 'NONE',  ( -6.900000000000019007, 2.500000000000000000, -4.676537180435978769 ) ) ;
#23780=ORIENTED_EDGE ( 'NONE', *, *, #46249, .F. ) ;
#23781=AXIS2_PLACEMENT_3D ( 'NONE', #31213, #41685, #101874 ) ;
#23782=EDGE_LOOP ( 'NONE', ( #36675, #103451, #104354, #55718 ) ) ;
#23783=AXIS2_PLACEMENT_3D ( 'NONE', #8042, #127823, #108816 ) ;
#23784=CARTESIAN_POINT ( 'NONE',  ( 12.49999999999993960, 2.500000000000000000, -4.330127018922201643 ) ) ;
#23785=DIRECTION ( 'NONE',  ( -0.000000000000000000, -1.000000000000000000, -0.000000000000000000 ) ) ;
#23786=CIRCLE ( 'NONE', #7024, 0.06509327318403743123 ) ;
#23788=DIRECTION ( 'NONE',  ( 0.000000000000000000, -0.9999939076577903929, 0.003490651415223739937 ) ) ;
#23789=DIRECTION ( 'NONE',  ( 0.000000000000000000, 0.000000000000000000, 1.000000000000000000 ) ) ;
#23790=DIRECTION ( 'NONE',  ( -0.000000000000000000, -1.000000000000000000, -0.000000000000000000 ) ) ;
#23791=CONICAL_SURFACE ( 'NONE', #40532, 0.09999999999999982514, 0.003490658503988666988 ) ;
#23793=CIRCLE ( 'NONE', #57233, 0.09999999999999982514 ) ;
#23794=VERTEX_POINT ( 'NONE', #8593 ) ;
#23795=CIRCLE ( 'NONE', #42683, 0.06509327318403745899 ) ;
#23796=CONICAL_SURFACE ( 'NONE', #21735, 0.1000000000000002554, 0.003490658503988666988 ) ;
#23797=CARTESIAN_POINT ( 'NONE',  ( 7.299999999999924327, 2.500000000000000000, 0.3464101615137735735 ) ) ;
#23798=CARTESIAN_POINT ( 'NONE',  ( -11.05000000000000071, 12.50000000000000000, -2.511473670974873951 ) ) ;
#23799=DIRECTION ( 'NONE',  ( 0.000000000000000000, 0.000000000000000000, 1.000000000000000000 ) ) ;
#23800=EDGE_LOOP ( 'NONE', ( #87413, #106530 ) ) ;
#23801=DIRECTION ( 'NONE',  ( 0.000000000000000000, 1.000000000000000000, 0.000000000000000000 ) ) ;
#23802=EDGE_CURVE ( 'NONE', #55739, #36661, #62989, .T. ) ;
#23803=VERTEX_POINT ( 'NONE', #67514 ) ;
#23804=CIRCLE ( 'NONE', #57250, 0.09999999999999982514 ) ;
#23805=CIRCLE ( 'NONE', #90699, 0.1000000000000000472 ) ;
#23806=AXIS2_PLACEMENT_3D ( 'NONE', #65232, #5663, #45625 ) ;
#23807=DIRECTION ( 'NONE',  ( -4.274815082592931898E-19, -0.9999939076577903929, -0.003490651415223739937 ) ) ;
#23808=VECTOR ( 'NONE', #44785, 1000.000000000000000 ) ;
#23809=EDGE_LOOP ( 'NONE', ( #33744, #122302, #85066, #61673 ) ) ;
#23810=DIRECTION ( 'NONE',  ( 0.000000000000000000, 0.000000000000000000, 1.000000000000000000 ) ) ;
#23811=CARTESIAN_POINT ( 'NONE',  ( -3.350000000000028955, 2.500000000000000000, 5.902370205355745192 ) ) ;
#23812=CARTESIAN_POINT ( 'NONE',  ( 8.949999999999915801, 12.50000000000000000, -1.818653347947326138 ) ) ;
#23813=CIRCLE ( 'NONE', #115734, 0.1000000000000002554 ) ;
#23814=ORIENTED_EDGE ( 'NONE', *, *, #50107, .T. ) ;
#23815=DIRECTION ( 'NONE',  ( -4.274815082592931898E-19, -0.9999939076577903929, -0.003490651415223739937 ) ) ;
#23817=ADVANCED_FACE ( 'NONE', ( #78665 ), #127738, .T. ) ;
#23818=ADVANCED_FACE ( 'NONE', ( #87167 ), #104733, .T. ) ;
#23819=VERTEX_POINT ( 'NONE', #28263 ) ;
#23820=ORIENTED_EDGE ( 'NONE', *, *, #42016, .T. ) ;
#23821=EDGE_LOOP ( 'NONE', ( #62367, #67228 ) ) ;
#23822=DIRECTION ( 'NONE',  ( 0.000000000000000000, -0.000000000000000000, 1.000000000000000000 ) ) ;
#23823=PLANE ( 'NONE',  #33360 ) ;
#23824=CIRCLE ( 'NONE', #124166, 0.06509327318403741736 ) ;
#23825=CARTESIAN_POINT ( 'NONE',  ( 10.84999999999991260, 2.500000000000000000, -1.572243186433550211 ) ) ;
#23826=CIRCLE ( 'NONE', #94830, 0.1000000000000002554 ) ;
#23827=EDGE_CURVE ( 'NONE', #51156, #4055, #2328, .T. ) ;
#23828=ORIENTED_EDGE ( 'NONE', *, *, #73366, .T. ) ;
#23829=DIRECTION ( 'NONE',  ( -0.000000000000000000, 1.000000000000000000, -0.000000000000000000 ) ) ;
#23830=DIRECTION ( 'NONE',  ( -0.000000000000000000, 1.000000000000000000, -0.000000000000000000 ) ) ;
#23831=ORIENTED_EDGE ( 'NONE', *, *, #59367, .T. ) ;
#23832=DIRECTION ( 'NONE',  ( 0.000000000000000000, 0.000000000000000000, 1.000000000000000000 ) ) ;
#23833=VECTOR ( 'NONE', #120711, 1000.000000000000000 ) ;
#23834=CARTESIAN_POINT ( 'NONE',  ( 0.8499999999999545697, 2.500000000000000000, 2.957883832488649389 ) ) ;
#23835=AXIS2_PLACEMENT_3D ( 'NONE', #22651, #84777, #44194 ) ;
#23836=AXIS2_PLACEMENT_3D ( 'NONE', #121986, #12016, #62433 ) ;
#23837=CIRCLE ( 'NONE', #80076, 0.06509327318403745899 ) ;
#23838=DIRECTION ( 'NONE',  ( 0.000000000000000000, 0.000000000000000000, 1.000000000000000000 ) ) ;
#23839=CONICAL_SURFACE ( 'NONE', #86219, 0.1000000000000002554, 0.003490658503988666988 ) ;
#23840=DIRECTION ( 'NONE',  ( 0.000000000000000000, 0.000000000000000000, 1.000000000000000000 ) ) ;
#23841=DIRECTION ( 'NONE',  ( 0.000000000000000000, 0.000000000000000000, 1.000000000000000000 ) ) ;
#23842=DIRECTION ( 'NONE',  ( 0.000000000000000000, 1.000000000000000000, 0.000000000000000000 ) ) ;
#23843=DIRECTION ( 'NONE',  ( -0.000000000000000000, 1.000000000000000000, -0.000000000000000000 ) ) ;
#23844=CIRCLE ( 'NONE', #76071, 0.1000000000000002554 ) ;
#23845=VECTOR ( 'NONE', #114521, 1000.000000000000000 ) ;
#23846=AXIS2_PLACEMENT_3D ( 'NONE', #43964, #110750, #61008 ) ;
#23847=EDGE_LOOP ( 'NONE', ( #48447, #20004 ) ) ;
#23848=ORIENTED_EDGE ( 'NONE', *, *, #36355, .F. ) ;
#23849=EDGE_LOOP ( 'NONE', ( #6645, #126955, #127097, #19229 ) ) ;
#23850=ORIENTED_EDGE ( 'NONE', *, *, #19014, .T. ) ;
#23851=FACE_OUTER_BOUND ( 'NONE', #90131, .T. ) ;
#23852=CARTESIAN_POINT ( 'NONE',  ( -12.29999999999999716, 2.500000000000000000, 0.2464101615137776757 ) ) ;
#23853=CIRCLE ( 'NONE', #67751, 0.06509327318403745899 ) ;
#23854=CARTESIAN_POINT ( 'NONE',  ( 3.099999999999943245, 2.500000000000000000, 3.883716857408420431 ) ) ;
#23855=ORIENTED_EDGE ( 'NONE', *, *, #22969, .T. ) ;
#23856=FACE_BOUND ( 'NONE', #47833, .T. ) ;
#23857=CARTESIAN_POINT ( 'NONE',  ( 2.699999999999944666, 2.500000000000000000, 4.776537180435972196 ) ) ;
#23858=CARTESIAN_POINT ( 'NONE',  ( 2.899999999999945732, 12.50000000000000000, -0.06509327318403980434 ) ) ;
#23859=DIRECTION ( 'NONE',  ( 0.000000000000000000, 0.000000000000000000, 1.000000000000000000 ) ) ;
#23860=ADVANCED_FACE ( 'NONE', ( #47268 ), #8587, .T. ) ;
#23861=DIRECTION ( 'NONE',  ( 0.000000000000000000, 0.000000000000000000, 1.000000000000000000 ) ) ;
#23862=DIRECTION ( 'NONE',  ( 0.000000000000000000, 0.000000000000000000, 1.000000000000000000 ) ) ;
#23863=CIRCLE ( 'NONE', #101219, 0.09999999999999982514 ) ;
#23864=DIRECTION ( 'NONE',  ( 0.000000000000000000, 1.000000000000000000, 0.000000000000000000 ) ) ;
#23865=DIRECTION ( 'NONE',  ( -0.000000000000000000, -1.000000000000000000, -0.000000000000000000 ) ) ;
#23866=DIRECTION ( 'NONE',  ( 0.000000000000000000, 0.000000000000000000, 1.000000000000000000 ) ) ;
#23867=EDGE_CURVE ( 'NONE', #41297, #32010, #38756, .T. ) ;
#23868=FACE_OUTER_BOUND ( 'NONE', #86326, .T. ) ;
#23869=EDGE_CURVE ( 'NONE', #29869, #67997, #52523, .T. ) ;
#23870=CIRCLE ( 'NONE', #97014, 0.06509327318403745899 ) ;
#23871=LINE ( 'NONE', #85352, #100410 ) ;
#23872=ORIENTED_EDGE ( 'NONE', *, *, #116127, .F. ) ;
#23873=ORIENTED_EDGE ( 'NONE', *, *, #93295, .F. ) ;
#23874=ORIENTED_EDGE ( 'NONE', *, *, #82182, .T. ) ;
#23875=ORIENTED_EDGE ( 'NONE', *, *, #25692, .T. ) ;
#23876=ORIENTED_EDGE ( 'NONE', *, *, #44116, .T. ) ;
#23877=EDGE_CURVE ( 'NONE', #39515, #6261, #81755, .T. ) ;
#23878=ORIENTED_EDGE ( 'NONE', *, *, #121367, .F. ) ;
#23879=DIRECTION ( 'NONE',  ( -0.000000000000000000, -1.000000000000000000, -0.000000000000000000 ) ) ;
#23880=EDGE_CURVE ( 'NONE', #56128, #4802, #98936, .T. ) ;
#23881=EDGE_CURVE ( 'NONE', #100348, #26373, #69229, .T. ) ;
#23882=ORIENTED_EDGE ( 'NONE', *, *, #33497, .T. ) ;
#23883=ORIENTED_EDGE ( 'NONE', *, *, #23639, .T. ) ;
#23884=AXIS2_PLACEMENT_3D ( 'NONE', #53143, #80362, #10932 ) ;
#23885=VECTOR ( 'NONE', #85137, 1000.000000000000000 ) ;
#23886=EDGE_CURVE ( 'NONE', #79541, #57283, #47912, .T. ) ;
#23887=CARTESIAN_POINT ( 'NONE',  ( 15.22989033483591470, -1.499999999999968470, 7.180069493258844915 ) ) ;
#23889=LINE ( 'NONE', #103734, #96933 ) ;
#23890=EDGE_LOOP ( 'NONE', ( #113371, #44265 ) ) ;
#23891=DIRECTION ( 'NONE',  ( -0.000000000000000000, 1.000000000000000000, -0.000000000000000000 ) ) ;
#23892=EDGE_CURVE ( 'NONE', #19348, #117873, #36805, .T. ) ;
#23893=ORIENTED_EDGE ( 'NONE', *, *, #45187, .F. ) ;
#23894=CIRCLE ( 'NONE', #44821, 0.1000000000000002554 ) ;
#23895=ORIENTED_EDGE ( 'NONE', *, *, #94026, .T. ) ;
#23896=CARTESIAN_POINT ( 'NONE',  ( 2.899999999999945732, 2.500000000000000000, -4.430127018922202176 ) ) ;
#23897=ORIENTED_EDGE ( 'NONE', *, *, #71898, .T. ) ;
#23899=VERTEX_POINT ( 'NONE', #78002 ) ;
#23900=DIRECTION ( 'NONE',  ( 0.000000000000000000, 1.000000000000000000, 0.000000000000000000 ) ) ;
#23901=DIRECTION ( 'NONE',  ( -0.000000000000000000, 1.000000000000000000, -0.000000000000000000 ) ) ;
#23902=AXIS2_PLACEMENT_3D ( 'NONE', #102838, #53120, #3366 ) ;
#23903=CARTESIAN_POINT ( 'NONE',  ( -1.900000000000034994, 2.500000000000000000, -0.4464101615137783252 ) ) ;
#23904=AXIS2_PLACEMENT_3D ( 'NONE', #58441, #39461, #68881 ) ;
#23905=CARTESIAN_POINT ( 'NONE',  ( 1.649999999999950617, 2.500000000000000000, 2.065063509461097624 ) ) ;
#23908=ORIENTED_EDGE ( 'NONE', *, *, #111178, .F. ) ;
#23909=AXIS2_PLACEMENT_3D ( 'NONE', #22063, #13498, #112368 ) ;
#23911=ORIENTED_EDGE ( 'NONE', *, *, #33062, .T. ) ;
#23912=CARTESIAN_POINT ( 'NONE',  ( 87.50000000000002842, 4.871203238224194543, 5.733266569811710234 ) ) ;
#23913=EDGE_LOOP ( 'NONE', ( #7529, #121263 ) ) ;
#23914=DIRECTION ( 'NONE',  ( 0.000000000000000000, -0.9999939076577903929, 0.003490651415223739937 ) ) ;
#23915=PLANE ( 'NONE',  #115846 ) ;
#23916=FACE_OUTER_BOUND ( 'NONE', #70140, .T. ) ;
#23917=DIRECTION ( 'NONE',  ( 0.000000000000000000, 0.000000000000000000, 1.000000000000000000 ) ) ;
#23918=ORIENTED_EDGE ( 'NONE', *, *, #58639, .F. ) ;
#23919=DIRECTION ( 'NONE',  ( 0.000000000000000000, 1.000000000000000000, 0.000000000000000000 ) ) ;
#23920=ADVANCED_FACE ( 'NONE', ( #79311 ), #44197, .T. ) ;
#23921=CIRCLE ( 'NONE', #42723, 0.06509327318403745899 ) ;
#23922=DIRECTION ( 'NONE',  ( 0.000000000000000000, 1.000000000000000000, 0.000000000000000000 ) ) ;
#23923=ORIENTED_EDGE ( 'NONE', *, *, #125004, .F. ) ;
#23924=EDGE_LOOP ( 'NONE', ( #122711, #47616 ) ) ;
#23925=AXIS2_PLACEMENT_3D ( 'NONE', #98571, #110347, #39061 ) ;
#23926=AXIS2_PLACEMENT_3D ( 'NONE', #22112, #92104, #32579 ) ;
#23927=VERTEX_POINT ( 'NONE', #48551 ) ;
#23928=DIRECTION ( 'NONE',  ( -0.000000000000000000, 1.000000000000000000, -0.000000000000000000 ) ) ;
#23929=DIRECTION ( 'NONE',  ( 0.000000000000000000, 1.000000000000000000, 0.000000000000000000 ) ) ;
#23931=DIRECTION ( 'NONE',  ( -1.000000000000000000, -0.000000000000000000, -0.000000000000000000 ) ) ;
#23932=EDGE_CURVE ( 'NONE', #125419, #43068, #21213, .T. ) ;
#23933=AXIS2_PLACEMENT_3D ( 'NONE', #87853, #106849, #27025 ) ;
#23934=AXIS2_PLACEMENT_3D ( 'NONE', #60139, #20837, #99404 ) ;
#23935=CARTESIAN_POINT ( 'NONE',  ( 17.34778429999903082, 2.317753570193296309, -4.873671836816706460 ) ) ;
#23936=CONICAL_SURFACE ( 'NONE', #55325, 0.1000000000000000472, 0.003490658503988666988 ) ;
#23937=DIRECTION ( 'NONE',  ( 0.000000000000000000, -0.000000000000000000, 1.000000000000000000 ) ) ;
#23938=ORIENTED_EDGE ( 'NONE', *, *, #52943, .F. ) ;
#23939=CIRCLE ( 'NONE', #55329, 0.06509327318403745899 ) ;
#23940=DIRECTION ( 'NONE',  ( -4.274815082592931898E-19, -0.9999939076577903929, -0.003490651415223739937 ) ) ;
#23941=EDGE_LOOP ( 'NONE', ( #37812, #32547 ) ) ;
#23942=DIRECTION ( 'NONE',  ( 0.000000000000000000, 1.000000000000000000, 0.000000000000000000 ) ) ;
#23943=CARTESIAN_POINT ( 'NONE',  ( -7.499999999999976907, 2.500000000000000000, 4.230127018922196669 ) ) ;
#23944=FACE_OUTER_BOUND ( 'NONE', #125431, .T. ) ;
#23945=DIRECTION ( 'NONE',  ( 0.000000000000000000, 0.000000000000000000, -1.000000000000000000 ) ) ;
#23946=ORIENTED_EDGE ( 'NONE', *, *, #101432, .F. ) ;
#23947=FACE_OUTER_BOUND ( 'NONE', #98465, .T. ) ;
#23948=CARTESIAN_POINT ( 'NONE',  ( -12.04999999999999538, 2.500000000000000000, 2.165063509461097713 ) ) ;
#23949=ORIENTED_EDGE ( 'NONE', *, *, #123992, .T. ) ;
#23950=VECTOR ( 'NONE', #56426, 1000.000000000000000 ) ;
#23951=ORIENTED_EDGE ( 'NONE', *, *, #45296, .T. ) ;
#23952=FACE_OUTER_BOUND ( 'NONE', #1428, .T. ) ;
#23953=EDGE_CURVE ( 'NONE', #109941, #13735, #106883, .T. ) ;
#23954=VERTEX_POINT ( 'NONE', #128422 ) ;
#23955=ORIENTED_EDGE ( 'NONE', *, *, #54605, .F. ) ;
#23956=DIRECTION ( 'NONE',  ( -4.274815082592931898E-19, -0.9999939076577903929, -0.003490651415223739937 ) ) ;
#23957=VERTEX_POINT ( 'NONE', #69456 ) ;
#23958=CARTESIAN_POINT ( 'NONE',  ( 15.05551045036142277, 2.483581587658090672, -4.666934263335500432 ) ) ;
#23959=LINE ( 'NONE', #54060, #109080 ) ;
#23960=CIRCLE ( 'NONE', #86652, 0.06509327318403745899 ) ;
#23961=DIRECTION ( 'NONE',  ( -0.000000000000000000, 1.000000000000000000, -0.000000000000000000 ) ) ;
#23963=VECTOR ( 'NONE', #129610, 1000.000000000000000 ) ;
#23964=EDGE_LOOP ( 'NONE', ( #18882, #706 ) ) ;
#23965=CARTESIAN_POINT ( 'NONE',  ( -8.550000000000011369, 2.500000000000000000, -2.411473670974877859 ) ) ;
#23966=LINE ( 'NONE', #14123, #50033 ) ;
#23967=VERTEX_POINT ( 'NONE', #14868 ) ;
#23968=EDGE_CURVE ( 'NONE', #79506, #51796, #25316, .T. ) ;
#23969=DIRECTION ( 'NONE',  ( -4.274815082592931898E-19, -0.9999939076577903929, -0.003490651415223739937 ) ) ;
#23970=CARTESIAN_POINT ( 'NONE',  ( -1.650000000000035660, 12.50000000000000000, 2.857883832488649301 ) ) ;
#23971=ADVANCED_FACE ( 'NONE', ( #100225 ), #110993, .T. ) ;
#23972=ORIENTED_EDGE ( 'NONE', *, *, #102582, .T. ) ;
#23973=VECTOR ( 'NONE', #125848, 1000.000000000000000 ) ;
#23974=VERTEX_POINT ( 'NONE', #79 ) ;
#23976=VECTOR ( 'NONE', #57650, 1000.000000000000000 ) ;
#23977=EDGE_LOOP ( 'NONE', ( #57395, #111708, #20440, #108121 ) ) ;
#23978=EDGE_LOOP ( 'NONE', ( #75175, #27062 ) ) ;
#23979=CARTESIAN_POINT ( 'NONE',  ( -11.24999999999996447, 2.500000000000000000, -6.495190528383298911 ) ) ;
#23980=DIRECTION ( 'NONE',  ( 0.000000000000000000, 0.000000000000000000, 1.000000000000000000 ) ) ;
#23981=DIRECTION ( 'NONE',  ( 0.000000000000000000, 1.000000000000000000, 0.000000000000000000 ) ) ;
#23982=ADVANCED_FACE ( 'NONE', ( #1362 ), #14838, .T. ) ;
#23983=FACE_BOUND ( 'NONE', #36376, .T. ) ;
#23984=ORIENTED_EDGE ( 'NONE', *, *, #28127, .F. ) ;
#23986=DIRECTION ( 'NONE',  ( 0.000000000000000000, 0.000000000000000000, -1.000000000000000000 ) ) ;
#23987=FACE_OUTER_BOUND ( 'NONE', #6956, .T. ) ;
#23988=FACE_OUTER_BOUND ( 'NONE', #12036, .T. ) ;
#23989=CARTESIAN_POINT ( 'NONE',  ( -3.750000000000027978, 2.500000000000000000, 7.088010851410848190 ) ) ;
#23990=CIRCLE ( 'NONE', #61364, 0.1000000000000000472 ) ;
#23991=CARTESIAN_POINT ( 'NONE',  ( -6.900000000000015454, 2.500000000000000000, 3.983716857408420076 ) ) ;
#23992=CIRCLE ( 'NONE', #72030, 0.1000000000000002554 ) ;
#23993=DIRECTION ( 'NONE',  ( 0.000000000000000000, 1.000000000000000000, 0.000000000000000000 ) ) ;
#23994=ORIENTED_EDGE ( 'NONE', *, *, #59202, .T. ) ;
#23995=ORIENTED_EDGE ( 'NONE', *, *, #53424, .T. ) ;
#23996=ORIENTED_EDGE ( 'NONE', *, *, #85012, .F. ) ;
#23997=ORIENTED_EDGE ( 'NONE', *, *, #95400, .F. ) ;
#23998=EDGE_LOOP ( 'NONE', ( #23938, #26795 ) ) ;
#23999=FACE_OUTER_BOUND ( 'NONE', #26931, .T. ) ;
#24000=CARTESIAN_POINT ( 'NONE',  ( 8.549999999999920774, 2.500000000000000000, -2.611473670974877592 ) ) ;
#24001=VERTEX_POINT ( 'NONE', #124214 ) ;
#24002=FACE_BOUND ( 'NONE', #41213, .T. ) ;
#24003=DIRECTION ( 'NONE',  ( 0.000000000000000000, 1.000000000000000000, 0.000000000000000000 ) ) ;
#24004=EDGE_CURVE ( 'NONE', #41537, #95313, #83653, .T. ) ;
#24005=CIRCLE ( 'NONE', #7255, 0.06509327318403745899 ) ;
#24006=CIRCLE ( 'NONE', #122212, 0.09999999999999982514 ) ;
#24007=VERTEX_POINT ( 'NONE', #120511 ) ;
#24008=AXIS2_PLACEMENT_3D ( 'NONE', #103231, #105146, #13545 ) ;
#24009=CARTESIAN_POINT ( 'NONE',  ( 105.5000000000000142, 0.000000000000000000, 0.000000000000000000 ) ) ;
#24010=CARTESIAN_POINT ( 'NONE',  ( -10.40000000000000391, 12.50000000000000000, -3.637306695894645614 ) ) ;
#24011=DIRECTION ( 'NONE',  ( 0.000000000000000000, 0.000000000000000000, 1.000000000000000000 ) ) ;
#24012=ORIENTED_EDGE ( 'NONE', *, *, #50547, .T. ) ;
#24013=CARTESIAN_POINT ( 'NONE',  ( -4.200000000000025935, 2.500000000000000000, -2.385244779468109755E-15 ) ) ;
#24014=ADVANCED_FACE ( 'NONE', ( #113760 ), #50463, .T. ) ;
#24015=AXIS2_PLACEMENT_3D ( 'NONE', #100373, #50615, #90539 ) ;
#24016=ORIENTED_EDGE ( 'NONE', *, *, #51526, .T. ) ;
#24017=AXIS2_PLACEMENT_3D ( 'NONE', #126250, #45120, #55577 ) ;
#24018=ORIENTED_EDGE ( 'NONE', *, *, #126087, .F. ) ;
#24019=VERTEX_POINT ( 'NONE', #33902 ) ;
#24020=ADVANCED_FACE ( 'NONE', ( #121147 ), #54193, .T. ) ;
#24021=CARTESIAN_POINT ( 'NONE',  ( 5.399999999999936406, 2.500000000000000000, -3.637306695894650055 ) ) ;
#24022=CIRCLE ( 'NONE', #82610, 0.09999999999999982514 ) ;
#24023=DIRECTION ( 'NONE',  ( -0.000000000000000000, -1.000000000000000000, -0.000000000000000000 ) ) ;
#24024=CARTESIAN_POINT ( 'NONE',  ( 10.39999999999991154, 12.50000000000000000, 3.572213422710607489 ) ) ;
#24025=EDGE_CURVE ( 'NONE', #81317, #72217, #21009, .T. ) ;
#24026=ORIENTED_EDGE ( 'NONE', *, *, #44976, .F. ) ;
#24027=CARTESIAN_POINT ( 'NONE',  ( 12.89999999999990266, 2.500000000000000000, 5.022947341949748790 ) ) ;
#24028=ADVANCED_FACE ( 'NONE', ( #3795 ), #23425, .T. ) ;
#24029=CONICAL_SURFACE ( 'NONE', #107650, 0.09999999999999982514, 0.003490658503988666988 ) ;
#24030=AXIS2_PLACEMENT_3D ( 'NONE', #10771, #11446, #16874 ) ;
#24031=CARTESIAN_POINT ( 'NONE',  ( -11.44999999999999751, 2.500000000000000000, 6.841600689897072485 ) ) ;
#24032=CARTESIAN_POINT ( 'NONE',  ( -7.500000000000015099, 12.50000000000000000, -5.088040615133791356 ) ) ;
#24033=EDGE_CURVE ( 'NONE', #94365, #117010, #92217, .T. ) ;
#24034=DIRECTION ( 'NONE',  ( 0.000000000000000000, -0.000000000000000000, 1.000000000000000000 ) ) ;
#24035=CONICAL_SURFACE ( 'NONE', #118012, 0.1000000000000002554, 0.003490658503988666988 ) ;
#24036=VERTEX_POINT ( 'NONE', #81231 ) ;
#24037=DIRECTION ( 'NONE',  ( 0.000000000000000000, 0.000000000000000000, 1.000000000000000000 ) ) ;
#24038=ORIENTED_EDGE ( 'NONE', *, *, #31428, .T. ) ;
#24039=CARTESIAN_POINT ( 'NONE',  ( 0.1999999999999571565, 2.500000000000000000, 3.983716857408420076 ) ) ;
#24040=EDGE_CURVE ( 'NONE', #71367, #4913, #79708, .T. ) ;
#24041=EDGE_CURVE ( 'NONE', #119467, #45959, #123609, .T. ) ;
#24042=EDGE_LOOP ( 'NONE', ( #58536, #101094, #28340, #93534 ) ) ;
#24043=ORIENTED_EDGE ( 'NONE', *, *, #115427, .F. ) ;
#24044=CARTESIAN_POINT ( 'NONE',  ( -6.450000000000016165, 2.500000000000000000, 2.411473670974873862 ) ) ;
#24045=DIRECTION ( 'NONE',  ( 0.000000000000000000, 0.000000000000000000, 1.000000000000000000 ) ) ;
#24046=PLANE ( 'NONE',  #15368 ) ;
#24047=DIRECTION ( 'NONE',  ( 0.000000000000000000, 0.000000000000000000, 1.000000000000000000 ) ) ;
#24049=ORIENTED_EDGE ( 'NONE', *, *, #77034, .F. ) ;
#24050=ORIENTED_EDGE ( 'NONE', *, *, #36034, .F. ) ;
#24051=CARTESIAN_POINT ( 'NONE',  ( 10.44999999999991402, 12.50000000000000000, -2.165063509461101710 ) ) ;
#24052=DIRECTION ( 'NONE',  ( -0.000000000000000000, -1.000000000000000000, -0.000000000000000000 ) ) ;
#24053=DIRECTION ( 'NONE',  ( 0.000000000000000000, -0.9999939076577903929, 0.003490651415223739937 ) ) ;
#24054=ORIENTED_EDGE ( 'NONE', *, *, #79409, .T. ) ;
#24056=CARTESIAN_POINT ( 'NONE',  ( -3.300000000000027800, 2.500000000000000000, -0.1000000000000022815 ) ) ;
#24057=AXIS2_PLACEMENT_3D ( 'NONE', #84050, #74894, #95175 ) ;
#24058=EDGE_LOOP ( 'NONE', ( #96539, #56752 ) ) ;
#24059=DIRECTION ( 'NONE',  ( 0.000000000000000000, 0.000000000000000000, -1.000000000000000000 ) ) ;
#24060=VECTOR ( 'NONE', #80340, 1000.000000000000000 ) ;
#24061=DIRECTION ( 'NONE',  ( 0.000000000000000000, 0.000000000000000000, 1.000000000000000000 ) ) ;
#24062=EDGE_LOOP ( 'NONE', ( #35587, #7662, #9192, #38991 ) ) ;
#24063=FACE_OUTER_BOUND ( 'NONE', #27302, .T. ) ;
#24064=FACE_OUTER_BOUND ( 'NONE', #20539, .T. ) ;
#24065=DIRECTION ( 'NONE',  ( 0.000000000000000000, 1.000000000000000000, 0.000000000000000000 ) ) ;
#24066=PLANE ( 'NONE',  #37546 ) ;
#24067=ORIENTED_EDGE ( 'NONE', *, *, #95407, .T. ) ;
#24068=CIRCLE ( 'NONE', #65910, 0.1000000000000002554 ) ;
#24069=DIRECTION ( 'NONE',  ( 0.000000000000000000, 0.000000000000000000, 1.000000000000000000 ) ) ;
#24070=ADVANCED_FACE ( 'NONE', ( #24727 ), #77642, .T. ) ;
#24071=DIRECTION ( 'NONE',  ( 0.000000000000000000, -0.9999939076577903929, 0.003490651415223739937 ) ) ;
#24072=AXIS2_PLACEMENT_3D ( 'NONE', #86283, #13683, #16248 ) ;
#24073=EDGE_LOOP ( 'NONE', ( #3929, #120563 ) ) ;
#24074=ORIENTED_EDGE ( 'NONE', *, *, #73601, .T. ) ;
#24076=DIRECTION ( 'NONE',  ( 0.000000000000000000, 0.000000000000000000, 1.000000000000000000 ) ) ;
#24077=DIRECTION ( 'NONE',  ( 0.000000000000000000, 0.000000000000000000, -1.000000000000000000 ) ) ;
#24078=DIRECTION ( 'NONE',  ( 0.000000000000000000, 0.000000000000000000, -1.000000000000000000 ) ) ;
#24079=CARTESIAN_POINT ( 'NONE',  ( -0.4500000000000402012, 2.500000000000000000, 2.165063509461097713 ) ) ;
#24080=EDGE_CURVE ( 'NONE', #43648, #3765, #40018, .T. ) ;
#24081=CONICAL_SURFACE ( 'NONE', #120220, 0.1000000000000002554, 0.003490658503988666988 ) ;
#24082=DIRECTION ( 'NONE',  ( -4.274815082592931898E-19, -0.9999939076577903929, -0.003490651415223739937 ) ) ;
#24083=AXIS2_PLACEMENT_3D ( 'NONE', #122061, #92592, #111585 ) ;
#24084=CARTESIAN_POINT ( 'NONE',  ( -8.100000000000010303, 12.50000000000000000, 3.983716857408420964 ) ) ;
#24085=DIRECTION ( 'NONE',  ( -0.000000000000000000, -1.000000000000000000, -0.000000000000000000 ) ) ;
#24086=DIRECTION ( 'NONE',  ( 0.000000000000000000, 1.000000000000000000, 0.000000000000000000 ) ) ;
#24087=DIRECTION ( 'NONE',  ( -4.274815082592931898E-19, -0.9999939076577903929, -0.003490651415223739937 ) ) ;
#24088=DIRECTION ( 'NONE',  ( 0.000000000000000000, 1.000000000000000000, 0.000000000000000000 ) ) ;
#24089=ORIENTED_EDGE ( 'NONE', *, *, #14077, .T. ) ;
#24090=EDGE_LOOP ( 'NONE', ( #44824, #72379, #101026, #126010 ) ) ;
#24091=ORIENTED_EDGE ( 'NONE', *, *, #111334, .T. ) ;
#24092=VERTEX_POINT ( 'NONE', #104568 ) ;
#24093=CIRCLE ( 'NONE', #11555, 0.06509327318403745899 ) ;
#24094=DIRECTION ( 'NONE',  ( 0.000000000000000000, 0.000000000000000000, 1.000000000000000000 ) ) ;
#24095=DIRECTION ( 'NONE',  ( 0.000000000000000000, -0.000000000000000000, 1.000000000000000000 ) ) ;
#24096=VERTEX_POINT ( 'NONE', #37764 ) ;
#24097=CARTESIAN_POINT ( 'NONE',  ( 6.249999999999968914, 12.50000000000000000, -6.560283801567339701 ) ) ;
#24098=DIRECTION ( 'NONE',  ( 0.000000000000000000, 1.000000000000000000, 0.000000000000000000 ) ) ;
#24099=LINE ( 'NONE', #52918, #64174 ) ;
#24100=ORIENTED_EDGE ( 'NONE', *, *, #49311, .T. ) ;
#24101=CIRCLE ( 'NONE', #97250, 0.09999999999999982514 ) ;
#24102=DIRECTION ( 'NONE',  ( 0.000000000000000000, 1.000000000000000000, 0.000000000000000000 ) ) ;
#24103=DIRECTION ( 'NONE',  ( 0.000000000000000000, 1.000000000000000000, 0.000000000000000000 ) ) ;
#24104=ORIENTED_EDGE ( 'NONE', *, *, #100965, .T. ) ;
#24105=CONICAL_SURFACE ( 'NONE', #86878, 0.1000000000000002554, 0.003490658503988666988 ) ;
#24107=AXIS2_PLACEMENT_3D ( 'NONE', #83323, #33577, #73474 ) ;
#24108=VERTEX_POINT ( 'NONE', #116307 ) ;
#24109=VERTEX_POINT ( 'NONE', #16802 ) ;
#24110=ORIENTED_EDGE ( 'NONE', *, *, #22204, .T. ) ;
#24111=CARTESIAN_POINT ( 'NONE',  ( 12.09999999999990550, 12.50000000000000000, 3.702399969078682407 ) ) ;
#24112=AXIS2_PLACEMENT_3D ( 'NONE', #35067, #24581, #23285 ) ;
#24114=DIRECTION ( 'NONE',  ( 0.000000000000000000, 1.000000000000000000, 0.000000000000000000 ) ) ;
#24115=CONICAL_SURFACE ( 'NONE', #17843, 0.09999999999999982514, 0.003490658503988666988 ) ;
#24116=DIRECTION ( 'NONE',  ( 0.000000000000000000, 1.000000000000000000, 0.000000000000000000 ) ) ;
#24117=CIRCLE ( 'NONE', #15778, 0.06509327318403745899 ) ;
#24118=EDGE_CURVE ( 'NONE', #94495, #115716, #73443, .T. ) ;
#24119=VERTEX_POINT ( 'NONE', #116950 ) ;
#24120=CARTESIAN_POINT ( 'NONE',  ( 9.549999999999915445, 2.500000000000000000, -2.165063509461101710 ) ) ;
#24121=ORIENTED_EDGE ( 'NONE', *, *, #67545, .T. ) ;
#24122=CARTESIAN_POINT ( 'NONE',  ( -0.2000000000000347888, 2.500000000000000000, 0.3464101615137758494 ) ) ;
#24123=CARTESIAN_POINT ( 'NONE',  ( 10.28037028451869084, -2.499999999999618527, -9.136909653094715367 ) ) ;
#24124=EDGE_CURVE ( 'NONE', #21163, #42755, #111076, .T. ) ;
#24125=EDGE_CURVE ( 'NONE', #95225, #119631, #66564, .T. ) ;
#24126=FACE_OUTER_BOUND ( 'NONE', #107497, .T. ) ;
#24127=CARTESIAN_POINT ( 'NONE',  ( 19.61395058415580905, -2.556813634648763767, 4.305699210823851431 ) ) ;
#24128=EDGE_CURVE ( 'NONE', #86700, #38783, #75746, .T. ) ;
#24129=ORIENTED_EDGE ( 'NONE', *, *, #61888, .T. ) ;
#24130=ORIENTED_EDGE ( 'NONE', *, *, #126274, .F. ) ;
#24131=ADVANCED_FACE ( 'NONE', ( #7645 ), #83989, .T. ) ;
#24132=EDGE_CURVE ( 'NONE', #43500, #97794, #97330, .T. ) ;
#24133=VERTEX_POINT ( 'NONE', #55479 ) ;
#24134=DIRECTION ( 'NONE',  ( 0.000000000000000000, 0.000000000000000000, 1.000000000000000000 ) ) ;
#24136=DIRECTION ( 'NONE',  ( -4.274815082592931898E-19, -0.9999939076577903929, -0.003490651415223739937 ) ) ;
#24137=ADVANCED_FACE ( 'NONE', ( #26661 ), #96664, .T. ) ;
#24138=FACE_BOUND ( 'NONE', #37199, .T. ) ;
#24139=CARTESIAN_POINT ( 'NONE',  ( 2.949999999999943334, 12.50000000000000000, 6.495190528383297135 ) ) ;
#24140=CIRCLE ( 'NONE', #118216, 0.1000000000000000056 ) ;
#24141=DIRECTION ( 'NONE',  ( 0.000000000000000000, 0.000000000000000000, 1.000000000000000000 ) ) ;
#24142=CARTESIAN_POINT ( 'NONE',  ( 9.149999999999915090, 12.50000000000000000, 6.495190528383297135 ) ) ;
#24144=AXIS2_PLACEMENT_3D ( 'NONE', #81331, #112725, #100952 ) ;
#24145=CARTESIAN_POINT ( 'NONE',  ( 8.549999999999924327, 12.50000000000000000, -6.841600689897077814 ) ) ;
#24147=ORIENTED_EDGE ( 'NONE', *, *, #19461, .F. ) ;
#24148=AXIS2_PLACEMENT_3D ( 'NONE', #57174, #17891, #97104 ) ;
#24149=AXIS2_PLACEMENT_3D ( 'NONE', #91435, #83563, #101256 ) ;
#24150=CARTESIAN_POINT ( 'NONE',  ( 7.499999999999960032, 12.50000000000000000, 0.06509327318403515528 ) ) ;
#24151=ORIENTED_EDGE ( 'NONE', *, *, #125367, .F. ) ;
#24152=VERTEX_POINT ( 'NONE', #47596 ) ;
#24153=ORIENTED_EDGE ( 'NONE', *, *, #40240, .T. ) ;
#24154=ORIENTED_EDGE ( 'NONE', *, *, #40411, .F. ) ;
#24155=DIRECTION ( 'NONE',  ( 0.000000000000000000, -0.000000000000000000, 1.000000000000000000 ) ) ;
#24156=FACE_BOUND ( 'NONE', #95139, .T. ) ;
#24157=PLANE ( 'NONE',  #34730 ) ;
#24158=AXIS2_PLACEMENT_3D ( 'NONE', #51033, #58906, #28806 ) ;
#24159=ORIENTED_EDGE ( 'NONE', *, *, #104424, .F. ) ;
#24160=FACE_OUTER_BOUND ( 'NONE', #19977, .T. ) ;
#24161=CARTESIAN_POINT ( 'NONE',  ( -0.6500000000000389910, 12.50000000000000000, -6.148780366869526226 ) ) ;
#24162=ORIENTED_EDGE ( 'NONE', *, *, #61807, .T. ) ;
#24163=DIRECTION ( 'NONE',  ( 0.000000000000000000, 1.000000000000000000, 0.000000000000000000 ) ) ;
#24164=DIRECTION ( 'NONE',  ( 0.000000000000000000, 0.000000000000000000, 1.000000000000000000 ) ) ;
#24165=CIRCLE ( 'NONE', #109854, 0.06509327318403745899 ) ;
#24166=AXIS2_PLACEMENT_3D ( 'NONE', #39501, #29653, #69566 ) ;
#24167=EDGE_CURVE ( 'NONE', #34349, #41184, #58882, .T. ) ;
#24168=ORIENTED_EDGE ( 'NONE', *, *, #128451, .F. ) ;
#24169=ADVANCED_FACE ( 'NONE', ( #86858 ), #71377, .T. ) ;
#24170=DIRECTION ( 'NONE',  ( 0.000000000000000000, 0.000000000000000000, 1.000000000000000000 ) ) ;
#24171=FACE_OUTER_BOUND ( 'NONE', #39006, .T. ) ;
#24172=ADVANCED_FACE ( 'NONE', ( #25348 ), #81848, .T. ) ;
#24173=ORIENTED_EDGE ( 'NONE', *, *, #115019, .T. ) ;
#24174=DIRECTION ( 'NONE',  ( 0.000000000000000000, -0.9999939076577903929, 0.003490651415223739937 ) ) ;
#24175=CARTESIAN_POINT ( 'NONE',  ( 10.44999999999991402, 2.500000000000000000, 6.395190528383296602 ) ) ;
#24176=AXIS2_PLACEMENT_3D ( 'NONE', #3742, #75070, #83610 ) ;
#24177=FACE_OUTER_BOUND ( 'NONE', #45699, .T. ) ;
#24178=EDGE_CURVE ( 'NONE', #129312, #127662, #123696, .T. ) ;
#24179=EDGE_CURVE ( 'NONE', #20597, #121932, #14921, .T. ) ;
#24180=ORIENTED_EDGE ( 'NONE', *, *, #41958, .F. ) ;
#24181=ORIENTED_EDGE ( 'NONE', *, *, #129083, .T. ) ;
#24182=DIRECTION ( 'NONE',  ( 0.000000000000000000, -0.9999939076577903929, 0.003490651415223739937 ) ) ;
#24183=CIRCLE ( 'NONE', #17912, 0.09999999999999982514 ) ;
#24184=ORIENTED_EDGE ( 'NONE', *, *, #100088, .T. ) ;
#24185=DIRECTION ( 'NONE',  ( 0.000000000000000000, 0.000000000000000000, 1.000000000000000000 ) ) ;
#24186=FACE_OUTER_BOUND ( 'NONE', #20519, .T. ) ;
#24187=EDGE_CURVE ( 'NONE', #9410, #35149, #40100, .T. ) ;
#24188=EDGE_CURVE ( 'NONE', #16690, #15822, #113248, .T. ) ;
#24189=AXIS2_PLACEMENT_3D ( 'NONE', #17217, #66342, #38186 ) ;
#24190=ORIENTED_EDGE ( 'NONE', *, *, #70582, .F. ) ;
#24191=CIRCLE ( 'NONE', #55492, 0.1000000000000002554 ) ;
#24192=PLANE ( 'NONE',  #97745 ) ;
#24193=DIRECTION ( 'NONE',  ( -0.000000000000000000, 1.000000000000000000, -0.000000000000000000 ) ) ;
#24194=DIRECTION ( 'NONE',  ( 0.000000000000000000, 0.000000000000000000, 1.000000000000000000 ) ) ;
#24196=CARTESIAN_POINT ( 'NONE',  ( 10.59999999999990905, 2.500000000000000000, -3.983716857408426293 ) ) ;
#24197=DIRECTION ( 'NONE',  ( 0.000000000000000000, -0.9999939076577903929, 0.003490651415223739937 ) ) ;
#24198=EDGE_CURVE ( 'NONE', #59055, #13197, #92319, .T. ) ;
#24199=AXIS2_PLACEMENT_3D ( 'NONE', #113910, #34720, #54970 ) ;
#24200=ORIENTED_EDGE ( 'NONE', *, *, #77814, .T. ) ;
#24201=ORIENTED_EDGE ( 'NONE', *, *, #109636, .F. ) ;
#24202=DIRECTION ( 'NONE',  ( -0.000000000000000000, -1.000000000000000000, -0.000000000000000000 ) ) ;
#24204=CONICAL_SURFACE ( 'NONE', #103628, 0.1000000000000000472, 0.003490658503988666988 ) ;
#24205=ORIENTED_EDGE ( 'NONE', *, *, #38781, .T. ) ;
#24206=ORIENTED_EDGE ( 'NONE', *, *, #123458, .T. ) ;
#24207=EDGE_LOOP ( 'NONE', ( #122225, #763, #7666, #36833 ) ) ;
#24208=PLANE ( 'NONE',  #35391 ) ;
#24209=CARTESIAN_POINT ( 'NONE',  ( 11.64999999999990443, 12.50000000000000000, -7.122917578226816815 ) ) ;
#24210=AXIS2_PLACEMENT_3D ( 'NONE', #105479, #66185, #5966 ) ;
#24211=CARTESIAN_POINT ( 'NONE',  ( 14.14999999999989377, 2.500000000000000000, -1.372243186433550033 ) ) ;
#24212=AXIS2_PLACEMENT_3D ( 'NONE', #83915, #83300, #44016 ) ;
#24214=FACE_OUTER_BOUND ( 'NONE', #66218, .T. ) ;
#24215=DIRECTION ( 'NONE',  ( 0.000000000000000000, 0.000000000000000000, -1.000000000000000000 ) ) ;
#24216=CARTESIAN_POINT ( 'NONE',  ( 21.24754738303277435, 0.7337760880902381988, 4.182111650399361835 ) ) ;
#24217=AXIS2_PLACEMENT_3D ( 'NONE', #96195, #108606, #66097 ) ;
#24218=DIRECTION ( 'NONE',  ( 0.000000000000000000, 1.000000000000000000, 0.000000000000000000 ) ) ;
#24219=DIRECTION ( 'NONE',  ( -0.000000000000000000, 1.000000000000000000, -0.000000000000000000 ) ) ;
#24220=DIRECTION ( 'NONE',  ( 0.000000000000000000, 0.000000000000000000, -1.000000000000000000 ) ) ;
#24221=ORIENTED_EDGE ( 'NONE', *, *, #81343, .F. ) ;
#24222=CARTESIAN_POINT ( 'NONE',  ( -1.650000000000034772, 2.500000000000000000, 2.165063509461097713 ) ) ;
#24223=ORIENTED_EDGE ( 'NONE', *, *, #97859, .F. ) ;
#24224=ORIENTED_EDGE ( 'NONE', *, *, #34103, .T. ) ;
#24225=CARTESIAN_POINT ( 'NONE',  ( -1.700000000000035261, 2.500000000000000000, 4.330127018922196314 ) ) ;
#24226=CARTESIAN_POINT ( 'NONE',  ( 10.39999999999991154, 2.500000000000000000, 4.922947341949748257 ) ) ;
#24227=AXIS2_PLACEMENT_3D ( 'NONE', #64097, #72642, #14334 ) ;
#24228=DIRECTION ( 'NONE',  ( -0.000000000000000000, -1.000000000000000000, -0.000000000000000000 ) ) ;
#24230=ADVANCED_FACE ( 'NONE', ( #45019 ), #364, .T. ) ;
#24232=CARTESIAN_POINT ( 'NONE',  ( 0.1999999999999636513, 12.50000000000000000, -0.3464101615137760715 ) ) ;
#24233=DIRECTION ( 'NONE',  ( 0.000000000000000000, 1.000000000000000000, 0.000000000000000000 ) ) ;
#24234=PLANE ( 'NONE',  #103274 ) ;
#24235=ORIENTED_EDGE ( 'NONE', *, *, #63851, .F. ) ;
#24236=CARTESIAN_POINT ( 'NONE',  ( -5.850000000000018296, 2.500000000000000000, 7.288010851410849256 ) ) ;
#24237=VECTOR ( 'NONE', #82471, 1000.000000000000000 ) ;
#24238=AXIS2_PLACEMENT_3D ( 'NONE', #63765, #23842, #103693 ) ;
#24239=DIRECTION ( 'NONE',  ( -4.274815082592931898E-19, -0.9999939076577903929, -0.003490651415223739937 ) ) ;
#24240=ORIENTED_EDGE ( 'NONE', *, *, #97600, .T. ) ;
#24241=ORIENTED_EDGE ( 'NONE', *, *, #79850, .T. ) ;
#24242=CIRCLE ( 'NONE', #97389, 0.1000000000000002554 ) ;
#24243=VERTEX_POINT ( 'NONE', #27942 ) ;
#24244=ORIENTED_EDGE ( 'NONE', *, *, #78946, .T. ) ;
#24245=CARTESIAN_POINT ( 'NONE',  ( -5.200000000000024158, 2.500000000000000000, -4.676537180435977881 ) ) ;
#24246=CARTESIAN_POINT ( 'NONE',  ( 13.09999999999989839, 2.500000000000000000, -0.3464101615137783474 ) ) ;
#24247=AXIS2_PLACEMENT_3D ( 'NONE', #122984, #54241, #94157 ) ;
#24248=CARTESIAN_POINT ( 'NONE',  ( 12.89999999999990088, 12.50000000000000000, 4.265033745738159077 ) ) ;
#24249=LINE ( 'NONE', #113925, #88364 ) ;
#24250=AXIS2_PLACEMENT_3D ( 'NONE', #96151, #7768, #5824 ) ;
#24251=VECTOR ( 'NONE', #30958, 1000.000000000000000 ) ;
#24252=DIRECTION ( 'NONE',  ( -0.000000000000000000, -1.000000000000000000, -0.000000000000000000 ) ) ;
#24254=FACE_OUTER_BOUND ( 'NONE', #21328, .T. ) ;
#24255=DIRECTION ( 'NONE',  ( -0.000000000000000000, 1.000000000000000000, -0.000000000000000000 ) ) ;
#24256=CARTESIAN_POINT ( 'NONE',  ( 2.499999999999945377, 12.50000000000000000, 5.022947341949748790 ) ) ;
#24257=VERTEX_POINT ( 'NONE', #124861 ) ;
#24258=ORIENTED_EDGE ( 'NONE', *, *, #67268, .T. ) ;
#24259=VERTEX_POINT ( 'NONE', #35204 ) ;
#24260=DIRECTION ( 'NONE',  ( 0.000000000000000000, 0.000000000000000000, 1.000000000000000000 ) ) ;
#24261=FACE_OUTER_BOUND ( 'NONE', #108872, .T. ) ;
#24262=DIRECTION ( 'NONE',  ( -4.274815082592931898E-19, -0.9999939076577903929, -0.003490651415223739937 ) ) ;
#24263=EDGE_CURVE ( 'NONE', #93088, #37898, #10852, .T. ) ;
#24264=VERTEX_POINT ( 'NONE', #29252 ) ;
#24265=DIRECTION ( 'NONE',  ( 0.000000000000000000, 0.000000000000000000, 1.000000000000000000 ) ) ;
#24266=DIRECTION ( 'NONE',  ( -0.000000000000000000, 1.000000000000000000, -0.000000000000000000 ) ) ;
#24267=EDGE_CURVE ( 'NONE', #116552, #11967, #118255, .T. ) ;
#24268=CARTESIAN_POINT ( 'NONE',  ( 13.54999999999990123, 2.500000000000000000, 1.918653347947321564 ) ) ;
#24269=DIRECTION ( 'NONE',  ( 0.000000000000000000, 1.000000000000000000, 0.000000000000000000 ) ) ;
#24270=EDGE_CURVE ( 'NONE', #79131, #16954, #120839, .T. ) ;
#24271=CIRCLE ( 'NONE', #114167, 0.1000000000000002554 ) ;
#24272=FACE_OUTER_BOUND ( 'NONE', #61933, .T. ) ;
#24273=VECTOR ( 'NONE', #41969, 1000.000000000000000 ) ;
#24274=ORIENTED_EDGE ( 'NONE', *, *, #79556, .T. ) ;
#24275=ADVANCED_FACE ( 'NONE', ( #69805 ), #39081, .T. ) ;
#24277=ORIENTED_EDGE ( 'NONE', *, *, #50038, .T. ) ;
#24278=EDGE_CURVE ( 'NONE', #36641, #43898, #28596, .T. ) ;
#24279=DIRECTION ( 'NONE',  ( 0.000000000000000000, -0.9999939076577903929, 0.003490651415223739937 ) ) ;
#24280=ADVANCED_FACE ( 'NONE', ( #58063 ), #17070, .T. ) ;
#24281=EDGE_CURVE ( 'NONE', #95824, #25449, #119506, .T. ) ;
#24282=CARTESIAN_POINT ( 'NONE',  ( 2.099999999999948574, 12.50000000000000000, 4.330127018922196314 ) ) ;
#24283=DIRECTION ( 'NONE',  ( -4.274815082592931898E-19, -0.9999939076577903929, -0.003490651415223739937 ) ) ;
#24284=DIRECTION ( 'NONE',  ( -0.000000000000000000, -1.000000000000000000, -0.000000000000000000 ) ) ;
#24285=AXIS2_PLACEMENT_3D ( 'NONE', #18620, #48740, #88652 ) ;
#24286=AXIS2_PLACEMENT_3D ( 'NONE', #88863, #37198, #67247 ) ;
#24287=LINE ( 'NONE', #94299, #52270 ) ;
#24288=VERTEX_POINT ( 'NONE', #41017 ) ;
#24289=ORIENTED_EDGE ( 'NONE', *, *, #16648, .F. ) ;
#24290=DIRECTION ( 'NONE',  ( -0.000000000000000000, 1.000000000000000000, -0.000000000000000000 ) ) ;
#24291=DIRECTION ( 'NONE',  ( 0.000000000000000000, 0.000000000000000000, 1.000000000000000000 ) ) ;
#24292=ADVANCED_FACE ( 'NONE', ( #88117 ), #100720, .T. ) ;
#24293=FACE_OUTER_BOUND ( 'NONE', #31451, .T. ) ;
#24294=DIRECTION ( 'NONE',  ( 0.000000000000000000, 0.000000000000000000, 1.000000000000000000 ) ) ;
#24295=ORIENTED_EDGE ( 'NONE', *, *, #112788, .T. ) ;
#24296=CIRCLE ( 'NONE', #74557, 0.09999999999999999167 ) ;
#24297=CONICAL_SURFACE ( 'NONE', #91197, 0.1000000000000002554, 0.003490658503988666988 ) ;
#24298=CARTESIAN_POINT ( 'NONE',  ( 1.649999999999950617, 12.50000000000000000, -2.165063509461101710 ) ) ;
#24299=EDGE_CURVE ( 'NONE', #26010, #42850, #80920, .T. ) ;
#24300=AXIS2_PLACEMENT_3D ( 'NONE', #55750, #17080, #57029 ) ;
#24301=CARTESIAN_POINT ( 'NONE',  ( 8.549999999999924327, 2.500000000000000000, -6.841600689897077814 ) ) ;
#24302=EDGE_LOOP ( 'NONE', ( #121389, #123177 ) ) ;
#24303=CARTESIAN_POINT ( 'NONE',  ( -9.350000000000006750, 2.500000000000000000, -1.818653347947325916 ) ) ;
#24304=ORIENTED_EDGE ( 'NONE', *, *, #71448, .T. ) ;
#24305=CARTESIAN_POINT ( 'NONE',  ( -6.050000000000022027, 12.50000000000000000, -6.148780366869526226 ) ) ;
#24306=VERTEX_POINT ( 'NONE', #98593 ) ;
#24307=CARTESIAN_POINT ( 'NONE',  ( -0.8500000000000382805, 2.500000000000000000, -2.857883832488653741 ) ) ;
#24308=DIRECTION ( 'NONE',  ( 0.000000000000000000, 0.000000000000000000, 1.000000000000000000 ) ) ;
#24309=ORIENTED_EDGE ( 'NONE', *, *, #50040, .F. ) ;
#24310=ORIENTED_EDGE ( 'NONE', *, *, #105416, .F. ) ;
#24312=DIRECTION ( 'NONE',  ( -0.000000000000000000, 1.000000000000000000, -0.000000000000000000 ) ) ;
#24313=AXIS2_PLACEMENT_3D ( 'NONE', #10948, #22755, #50919 ) ;
#24315=CARTESIAN_POINT ( 'NONE',  ( -0.6500000000000403233, 12.50000000000000000, 6.148780366869520009 ) ) ;
#24316=CONICAL_SURFACE ( 'NONE', #13838, 0.09999999999999982514, 0.003490658503988666988 ) ;
#24317=CARTESIAN_POINT ( 'NONE',  ( -6.850000000000013856, 2.500000000000000000, 6.148780366869520897 ) ) ;
#24318=DIRECTION ( 'NONE',  ( 0.000000000000000000, 1.000000000000000000, 0.000000000000000000 ) ) ;
#24319=FACE_OUTER_BOUND ( 'NONE', #121455, .T. ) ;
#24320=AXIS2_PLACEMENT_3D ( 'NONE', #108537, #88902, #78457 ) ;
#24321=EDGE_CURVE ( 'NONE', #81450, #14967, #71475, .T. ) ;
#24322=CARTESIAN_POINT ( 'NONE',  ( 1.249999999999952038, 12.50000000000000000, 5.802370205355744659 ) ) ;
#24323=AXIS2_PLACEMENT_3D ( 'NONE', #92087, #31263, #40445 ) ;
#24324=EDGE_CURVE ( 'NONE', #122022, #80208, #78350, .T. ) ;
#24325=AXIS2_PLACEMENT_3D ( 'NONE', #2733, #70842, #50545 ) ;
#24326=ORIENTED_EDGE ( 'NONE', *, *, #85896, .F. ) ;
#24327=CIRCLE ( 'NONE', #41078, 0.1000000000000000056 ) ;
#24328=ADVANCED_FACE ( 'NONE', ( #120200 ), #29882, .T. ) ;
#24329=ORIENTED_EDGE ( 'NONE', *, *, #64829, .T. ) ;
#24330=CARTESIAN_POINT ( 'NONE',  ( -3.350000000000028955, 12.50000000000000000, 2.165063509461097713 ) ) ;
#24331=FACE_OUTER_BOUND ( 'NONE', #32264, .T. ) ;
#24332=CARTESIAN_POINT ( 'NONE',  ( 4.999999999999935163, 12.50000000000000000, 3.637306695894644726 ) ) ;
#24333=DIRECTION ( 'NONE',  ( 0.000000000000000000, 1.000000000000000000, 0.000000000000000000 ) ) ;
#24334=ORIENTED_EDGE ( 'NONE', *, *, #83726, .T. ) ;
#24335=VERTEX_POINT ( 'NONE', #119534 ) ;
#24336=LINE ( 'NONE', #85815, #112274 ) ;
#24337=ORIENTED_EDGE ( 'NONE', *, *, #5042, .F. ) ;
#24338=ADVANCED_FACE ( 'NONE', ( #18763 ), #42153, .T. ) ;
#24339=PLANE ( 'NONE',  #19941 ) ;
#24340=CARTESIAN_POINT ( 'NONE',  ( 18.70618316909975221, -2.558637580971239611, 2.503050677946469182 ) ) ;
#24341=AXIS2_PLACEMENT_3D ( 'NONE', #105270, #45076, #74527 ) ;
#24342=ADVANCED_FACE ( 'NONE', ( #118901 ), #6605, .T. ) ;
#24343=ORIENTED_EDGE ( 'NONE', *, *, #128975, .T. ) ;
#24344=CARTESIAN_POINT ( 'NONE',  ( 2.499999999999947153, 2.500000000000000000, 3.737306695894644371 ) ) ;
#24345=PLANE ( 'NONE',  #22214 ) ;
#24346=DIRECTION ( 'NONE',  ( 0.000000000000000000, 0.000000000000000000, -1.000000000000000000 ) ) ;
#24347=VECTOR ( 'NONE', #120948, 1000.000000000000000 ) ;
#24348=AXIS2_PLACEMENT_3D ( 'NONE', #39340, #38021, #117854 ) ;
#24349=EDGE_CURVE ( 'NONE', #3070, #92934, #99276, .T. ) ;
#24350=FACE_OUTER_BOUND ( 'NONE', #105777, .T. ) ;
#24351=DIRECTION ( 'NONE',  ( -4.274815082592931898E-19, -0.9999939076577903929, -0.003490651415223739937 ) ) ;
#24352=DIRECTION ( 'NONE',  ( 0.000000000000000000, 0.000000000000000000, 1.000000000000000000 ) ) ;
#24353=DIRECTION ( 'NONE',  ( -0.000000000000000000, -1.000000000000000000, -0.000000000000000000 ) ) ;
#24354=DIRECTION ( 'NONE',  ( 0.000000000000000000, -0.9999939076577903929, 0.003490651415223739937 ) ) ;
#24355=CARTESIAN_POINT ( 'NONE',  ( 0.4499999999999569344, 2.500000000000000000, -2.065063509461102065 ) ) ;
#24356=EDGE_CURVE ( 'NONE', #22443, #26454, #48411, .T. ) ;
#24357=VERTEX_POINT ( 'NONE', #52103 ) ;
#24358=ORIENTED_EDGE ( 'NONE', *, *, #24187, .F. ) ;
#24359=VERTEX_POINT ( 'NONE', #32487 ) ;
#24360=CARTESIAN_POINT ( 'NONE',  ( -3.150000000000029665, 2.500000000000000000, 6.741600689897071952 ) ) ;
#24361=ORIENTED_EDGE ( 'NONE', *, *, #59767, .F. ) ;
#24362=VERTEX_POINT ( 'NONE', #1693 ) ;
#24363=ORIENTED_EDGE ( 'NONE', *, *, #1368, .T. ) ;
#24364=ORIENTED_EDGE ( 'NONE', *, *, #49351, .F. ) ;
#24365=CARTESIAN_POINT ( 'NONE',  ( 11.64999999999990621, 12.50000000000000000, -2.230156782645139391 ) ) ;
#24366=CARTESIAN_POINT ( 'NONE',  ( 10.64999999999991331, 2.500000000000000000, 6.941600689897073018 ) ) ;
#24368=DIRECTION ( 'NONE',  ( 0.000000000000000000, 0.000000000000000000, 1.000000000000000000 ) ) ;
#24369=CARTESIAN_POINT ( 'NONE',  ( -12.69999999999999396, 2.500000000000000000, 0.2464101615137776757 ) ) ;
#24370=EDGE_CURVE ( 'NONE', #16509, #98934, #21339, .T. ) ;
#24371=VERTEX_POINT ( 'NONE', #122773 ) ;
#24372=CARTESIAN_POINT ( 'NONE',  ( 10.39999999999991509, 2.500000000000000000, -0.6928203230275542523 ) ) ;
#24374=AXIS2_PLACEMENT_3D ( 'NONE', #77312, #108058, #119169 ) ;
#24375=ORIENTED_EDGE ( 'NONE', *, *, #11089, .T. ) ;
#24377=AXIS2_PLACEMENT_3D ( 'NONE', #75276, #115177, #55647 ) ;
#24378=CARTESIAN_POINT ( 'NONE',  ( -9.350000000000004974, 12.50000000000000000, 6.841600689897072485 ) ) ;
#24379=VERTEX_POINT ( 'NONE', #41659 ) ;
#24380=EDGE_LOOP ( 'NONE', ( #74689, #16497 ) ) ;
#24381=VERTEX_POINT ( 'NONE', #112313 ) ;
#24382=CARTESIAN_POINT ( 'NONE',  ( 10.59999999999990905, 2.500000000000000000, -3.883716857408426648 ) ) ;
#24383=AXIS2_PLACEMENT_3D ( 'NONE', #10564, #69490, #9295 ) ;
#24384=VECTOR ( 'NONE', #24635, 1000.000000000000000 ) ;
#24385=DIRECTION ( 'NONE',  ( 0.000000000000000000, 1.000000000000000000, 0.000000000000000000 ) ) ;
#24386=DIRECTION ( 'NONE',  ( 0.000000000000000000, 0.000000000000000000, 1.000000000000000000 ) ) ;
#24388=CARTESIAN_POINT ( 'NONE',  ( -8.100000000000013856, 2.500000000000000000, -0.3464101615137782364 ) ) ;
#24389=CARTESIAN_POINT ( 'NONE',  ( 6.249999999999967137, 2.500000000000000000, 6.495190528383297135 ) ) ;
#24390=FACE_OUTER_BOUND ( 'NONE', #117107, .T. ) ;
#24391=DIRECTION ( 'NONE',  ( 0.000000000000000000, 0.000000000000000000, 1.000000000000000000 ) ) ;
#24392=CIRCLE ( 'NONE', #34878, 0.06509327318403745899 ) ;
#24393=AXIS2_PLACEMENT_3D ( 'NONE', #93681, #43949, #84510 ) ;
#24394=VERTEX_POINT ( 'NONE', #51467 ) ;
#24395=DIRECTION ( 'NONE',  ( 0.000000000000000000, 0.000000000000000000, 1.000000000000000000 ) ) ;
#24398=ORIENTED_EDGE ( 'NONE', *, *, #61082, .F. ) ;
#24399=ADVANCED_FACE ( 'NONE', ( #113597 ), #14083, .T. ) ;
#24400=VERTEX_POINT ( 'NONE', #73023 ) ;
#24401=DIRECTION ( 'NONE',  ( 0.000000000000000000, -0.9999939076577903929, 0.003490651415223739937 ) ) ;
#24403=DIRECTION ( 'NONE',  ( 0.000000000000000000, 0.000000000000000000, -1.000000000000000000 ) ) ;
#24404=ORIENTED_EDGE ( 'NONE', *, *, #41220, .T. ) ;
#24405=DIRECTION ( 'NONE',  ( 0.000000000000000000, 1.000000000000000000, 0.000000000000000000 ) ) ;
#24406=ORIENTED_EDGE ( 'NONE', *, *, #47275, .F. ) ;
#24407=LINE ( 'NONE', #14570, #41512 ) ;
#24408=PLANE ( 'NONE',  #18021 ) ;
#24409=DIRECTION ( 'NONE',  ( 0.000000000000000000, 1.000000000000000000, 0.000000000000000000 ) ) ;
#24410=AXIS2_PLACEMENT_3D ( 'NONE', #6927, #105808, #6288 ) ;
#24411=LINE ( 'NONE', #23776, #55581 ) ;
#24412=CIRCLE ( 'NONE', #97561, 0.1000000000000002554 ) ;
#24413=CARTESIAN_POINT ( 'NONE',  ( -0.8500000000000395017, 12.50000000000000000, 2.165063509461097713 ) ) ;
#24414=ORIENTED_EDGE ( 'NONE', *, *, #90047, .F. ) ;
#24415=CONICAL_SURFACE ( 'NONE', #9747, 0.09999999999999999167, 0.003490658503988666988 ) ;
#24416=AXIS2_PLACEMENT_3D ( 'NONE', #41734, #39162, #120280 ) ;
#24417=EDGE_LOOP ( 'NONE', ( #114502, #113111 ) ) ;
#24418=CIRCLE ( 'NONE', #82919, 0.06509327318403745899 ) ;
#24419=CARTESIAN_POINT ( 'NONE',  ( 9.399999999999915090, 12.50000000000000000, -4.676537180435977881 ) ) ;
#24420=DIRECTION ( 'NONE',  ( 0.000000000000000000, 0.000000000000000000, 1.000000000000000000 ) ) ;
#24421=CIRCLE ( 'NONE', #99742, 0.06509327318403745899 ) ;
#24422=EDGE_CURVE ( 'NONE', #126052, #114688, #52735, .T. ) ;
#24424=CARTESIAN_POINT ( 'NONE',  ( -11.25000000000000000, 2.500000000000000000, 7.288010851410849256 ) ) ;
#24425=DIRECTION ( 'NONE',  ( 0.000000000000000000, 0.000000000000000000, -1.000000000000000000 ) ) ;
#24426=DIRECTION ( 'NONE',  ( 0.000000000000000000, 1.000000000000000000, 0.000000000000000000 ) ) ;
#24427=DIRECTION ( 'NONE',  ( 0.000000000000000000, -0.9999939076577903929, 0.003490651415223739937 ) ) ;
#24428=VERTEX_POINT ( 'NONE', #82207 ) ;
#24429=CONICAL_SURFACE ( 'NONE', #107963, 0.1000000000000002554, 0.003490658503988666988 ) ;
#24431=DIRECTION ( 'NONE',  ( 0.000000000000000000, 1.000000000000000000, 0.000000000000000000 ) ) ;
#24432=CIRCLE ( 'NONE', #41187, 0.06509327318403745899 ) ;
#24433=AXIS2_PLACEMENT_3D ( 'NONE', #94350, #4660, #44619 ) ;
#24434=DIRECTION ( 'NONE',  ( 0.000000000000000000, 1.000000000000000000, 0.000000000000000000 ) ) ;
#24435=DIRECTION ( 'NONE',  ( 0.000000000000000000, 1.000000000000000000, 0.000000000000000000 ) ) ;
#24436=EDGE_LOOP ( 'NONE', ( #110069, #128129 ) ) ;
#24437=EDGE_CURVE ( 'NONE', #65711, #54010, #54744, .T. ) ;
#24438=EDGE_CURVE ( 'NONE', #31853, #16422, #103129, .T. ) ;
#24439=ADVANCED_FACE ( 'NONE', ( #42953 ), #92509, .T. ) ;
#24440=ADVANCED_FACE ( 'NONE', ( #42283 ), #31988, .T. ) ;
#24441=CARTESIAN_POINT ( 'NONE',  ( -5.850000000000022737, 12.50000000000000000, -2.230156782645139391 ) ) ;
#24442=EDGE_LOOP ( 'NONE', ( #49303, #3888, #97712, #76884 ) ) ;
#24443=ADVANCED_FACE ( 'NONE', ( #61283 ), #86234, .T. ) ;
#24444=CARTESIAN_POINT ( 'NONE',  ( 1.649999999999951061, 2.500000000000000000, -6.395190528383301931 ) ) ;
#24445=EDGE_LOOP ( 'NONE', ( #80663, #29291, #98992, #6003 ) ) ;
#24446=CARTESIAN_POINT ( 'NONE',  ( 8.749999999999921840, 12.50000000000000000, -5.737276932171712751 ) ) ;
#24447=DIRECTION ( 'NONE',  ( 0.000000000000000000, 0.000000000000000000, -1.000000000000000000 ) ) ;
#24448=VECTOR ( 'NONE', #5654, 1000.000000000000000 ) ;
#24449=EDGE_CURVE ( 'NONE', #4367, #6762, #19436, .T. ) ;
#24450=DIRECTION ( 'NONE',  ( -0.000000000000000000, 1.000000000000000000, -0.000000000000000000 ) ) ;
#24451=EDGE_LOOP ( 'NONE', ( #122681, #112502 ) ) ;
#24452=EDGE_CURVE ( 'NONE', #15915, #92369, #69518, .T. ) ;
#24453=CARTESIAN_POINT ( 'NONE',  ( -3.100000000000028511, 12.50000000000000000, -3.983716857408426293 ) ) ;
#24454=ADVANCED_FACE ( 'NONE', ( #83504 ), #102485, .T. ) ;
#24455=DIRECTION ( 'NONE',  ( -0.000000000000000000, 1.000000000000000000, -0.000000000000000000 ) ) ;
#24456=EDGE_CURVE ( 'NONE', #29616, #34192, #117614, .T. ) ;
#24457=ORIENTED_EDGE ( 'NONE', *, *, #68644, .F. ) ;
#24458=CARTESIAN_POINT ( 'NONE',  ( 11.64999999999990443, 12.50000000000000000, -7.188010851410854052 ) ) ;
#24459=AXIS2_PLACEMENT_3D ( 'NONE', #101957, #128867, #50282 ) ;
#24460=ORIENTED_EDGE ( 'NONE', *, *, #115850, .T. ) ;
#24461=AXIS2_PLACEMENT_3D ( 'NONE', #106360, #96518, #6842 ) ;
#24462=VERTEX_POINT ( 'NONE', #91374 ) ;
#24463=DIRECTION ( 'NONE',  ( -4.274815082592931898E-19, -0.9999939076577903929, -0.003490651415223739937 ) ) ;
#24464=CARTESIAN_POINT ( 'NONE',  ( -3.950000000000026379, 12.50000000000000000, 2.511473670974873507 ) ) ;
#24465=CARTESIAN_POINT ( 'NONE',  ( 3.349999999999942801, 2.500000000000000000, 2.857883832488649301 ) ) ;
#24466=ORIENTED_EDGE ( 'NONE', *, *, #25859, .T. ) ;
#24467=DIRECTION ( 'NONE',  ( 0.000000000000000000, 0.000000000000000000, -1.000000000000000000 ) ) ;
#24468=CARTESIAN_POINT ( 'NONE',  ( -2.700000000000031264, 2.500000000000000000, 4.676537180435972552 ) ) ;
#24469=ORIENTED_EDGE ( 'NONE', *, *, #1538, .T. ) ;
#24470=CIRCLE ( 'NONE', #103892, 0.06509327318403745899 ) ;
#24471=AXIS2_PLACEMENT_3D ( 'NONE', #102648, #64022, #103950 ) ;
#24472=FACE_OUTER_BOUND ( 'NONE', #28764, .T. ) ;
#24473=FACE_OUTER_BOUND ( 'NONE', #101116, .T. ) ;
#24474=DIRECTION ( 'NONE',  ( 0.000000000000000000, -0.000000000000000000, 1.000000000000000000 ) ) ;
#24475=CARTESIAN_POINT ( 'NONE',  ( 4.549999999999939426, 2.500000000000000000, -2.165063509461101710 ) ) ;
#24476=DIRECTION ( 'NONE',  ( 0.000000000000000000, -0.9999939076577903929, 0.003490651415223739937 ) ) ;
#24477=CARTESIAN_POINT ( 'NONE',  ( -2.700000000000030376, 2.500000000000000000, 4.083716857408421497 ) ) ;
#24478=CARTESIAN_POINT ( 'NONE',  ( 10.59999999999990905, 2.500000000000000000, -4.676537180435978769 ) ) ;
#24479=AXIS2_PLACEMENT_3D ( 'NONE', #402, #30556, #55959 ) ;
#24480=AXIS2_PLACEMENT_3D ( 'NONE', #62157, #50380, #102066 ) ;
#24481=AXIS2_PLACEMENT_3D ( 'NONE', #104952, #63775, #64402 ) ;
#24482=ORIENTED_EDGE ( 'NONE', *, *, #78265, .T. ) ;
#24483=EDGE_LOOP ( 'NONE', ( #63828, #81850 ) ) ;
#24484=VERTEX_POINT ( 'NONE', #54032 ) ;
#24485=ORIENTED_EDGE ( 'NONE', *, *, #50010, .F. ) ;
#24486=CARTESIAN_POINT ( 'NONE',  ( 7.949999999999922018, 2.500000000000000000, 6.395190528383296602 ) ) ;
#24487=DIRECTION ( 'NONE',  ( 0.000000000000000000, -0.000000000000000000, 1.000000000000000000 ) ) ;
#24488=LINE ( 'NONE', #126560, #90704 ) ;
#24489=EDGE_LOOP ( 'NONE', ( #68978, #119574, #121638, #124222 ) ) ;
#24490=FACE_BOUND ( 'NONE', #13100, .T. ) ;
#24491=CARTESIAN_POINT ( 'NONE',  ( -10.85000000000000142, 2.500000000000000000, -6.495190528383298911 ) ) ;
#24492=DIRECTION ( 'NONE',  ( 0.000000000000000000, -0.9999939076577903929, 0.003490651415223739937 ) ) ;
#24493=ADVANCED_FACE ( 'NONE', ( #44195 ), #25705, .T. ) ;
#24495=CARTESIAN_POINT ( 'NONE',  ( 7.499999999999927169, 12.50000000000000000, 3.637306695894644726 ) ) ;
#24496=ADVANCED_FACE ( 'NONE', ( #116801 ), #77929, .T. ) ;
#24497=DIRECTION ( 'NONE',  ( 0.000000000000000000, 1.000000000000000000, 0.000000000000000000 ) ) ;
#24498=LINE ( 'NONE', #64416, #97664 ) ;
#24499=CARTESIAN_POINT ( 'NONE',  ( -0.6000000000000383915, 2.500000000000000000, -3.983716857408426293 ) ) ;
#24500=DIRECTION ( 'NONE',  ( 0.000000000000000000, 0.000000000000000000, 1.000000000000000000 ) ) ;
#24501=FACE_OUTER_BOUND ( 'NONE', #4649, .T. ) ;
#24502=CONICAL_SURFACE ( 'NONE', #20297, 0.1000000000000000056, 0.003490658503988666988 ) ;
#24503=VECTOR ( 'NONE', #13219, 1000.000000000000000 ) ;
#24504=CARTESIAN_POINT ( 'NONE',  ( -12.04999999999999538, 12.50000000000000000, 2.165063509461097713 ) ) ;
#24505=EDGE_CURVE ( 'NONE', #14107, #91704, #15218, .T. ) ;
#24506=ORIENTED_EDGE ( 'NONE', *, *, #13342, .F. ) ;
#24507=VECTOR ( 'NONE', #78061, 1000.000000000000000 ) ;
#24508=ORIENTED_EDGE ( 'NONE', *, *, #40424, .T. ) ;
#24509=EDGE_LOOP ( 'NONE', ( #41394, #1768 ) ) ;
#24510=ORIENTED_EDGE ( 'NONE', *, *, #87935, .F. ) ;
#24511=CARTESIAN_POINT ( 'NONE',  ( 13.94999999999989804, 2.500000000000000000, 1.818653347947321475 ) ) ;
#24513=CARTESIAN_POINT ( 'NONE',  ( -4.550000000000022915, 12.50000000000000000, 6.495190528383297135 ) ) ;
#24514=ORIENTED_EDGE ( 'NONE', *, *, #54871, .F. ) ;
#24515=CIRCLE ( 'NONE', #55896, 0.06509327318403741736 ) ;
#24516=ORIENTED_EDGE ( 'NONE', *, *, #58667, .F. ) ;
#24518=CONICAL_SURFACE ( 'NONE', #120662, 0.1000000000000002554, 0.003490658503988666988 ) ;
#24519=DIRECTION ( 'NONE',  ( -0.000000000000000000, -1.000000000000000000, -0.000000000000000000 ) ) ;
#24520=CARTESIAN_POINT ( 'NONE',  ( 3.299999999999942979, 2.500000000000000000, 4.330127018922196314 ) ) ;
#24521=DIRECTION ( 'NONE',  ( 0.000000000000000000, 0.000000000000000000, -1.000000000000000000 ) ) ;
#24522=DIRECTION ( 'NONE',  ( 0.000000000000000000, 1.000000000000000000, 0.000000000000000000 ) ) ;
#24523=AXIS2_PLACEMENT_3D ( 'NONE', #94220, #56221, #46400 ) ;
#24524=ORIENTED_EDGE ( 'NONE', *, *, #61194, .F. ) ;
#24525=ORIENTED_EDGE ( 'NONE', *, *, #39990, .F. ) ;
#24526=CONICAL_SURFACE ( 'NONE', #76757, 0.1000000000000002554, 0.003490658503988666988 ) ;
#24527=AXIS2_PLACEMENT_3D ( 'NONE', #61374, #68111, #1152 ) ;
#24528=ORIENTED_EDGE ( 'NONE', *, *, #91998, .F. ) ;
#24529=DIRECTION ( 'NONE',  ( 0.000000000000000000, 0.000000000000000000, 1.000000000000000000 ) ) ;
#24530=VERTEX_POINT ( 'NONE', #56585 ) ;
#24532=EDGE_LOOP ( 'NONE', ( #5488, #89716, #100803, #6643 ) ) ;
#24533=ORIENTED_EDGE ( 'NONE', *, *, #115171, .T. ) ;
#24534=DIRECTION ( 'NONE',  ( -0.000000000000000000, -1.000000000000000000, -0.000000000000000000 ) ) ;
#24535=PLANE ( 'NONE',  #83032 ) ;
#24536=DIRECTION ( 'NONE',  ( -0.000000000000000000, -1.000000000000000000, -0.000000000000000000 ) ) ;
#24537=FACE_OUTER_BOUND ( 'NONE', #96766, .T. ) ;
#24538=LINE ( 'NONE', #54627, #87913 ) ;
#24539=AXIS2_PLACEMENT_3D ( 'NONE', #97690, #37504, #88507 ) ;
#24541=DIRECTION ( 'NONE',  ( -4.274815082592931898E-19, -0.9999939076577903929, -0.003490651415223739937 ) ) ;
#24542=ORIENTED_EDGE ( 'NONE', *, *, #66849, .F. ) ;
#24543=CARTESIAN_POINT ( 'NONE',  ( 17.50000000000000000, 2.499999999999999556, 1.333333333333336590 ) ) ;
#24544=ORIENTED_EDGE ( 'NONE', *, *, #56789, .T. ) ;
#24545=FACE_OUTER_BOUND ( 'NONE', #55239, .T. ) ;
#24546=DIRECTION ( 'NONE',  ( -1.000000000000000000, 0.000000000000000000, 0.000000000000000000 ) ) ;
#24547=EDGE_CURVE ( 'NONE', #14028, #39660, #47439, .T. ) ;
#24548=FACE_OUTER_BOUND ( 'NONE', #67227, .T. ) ;
#24549=EDGE_CURVE ( 'NONE', #66106, #52738, #55326, .T. ) ;
#24550=DIRECTION ( 'NONE',  ( 0.000000000000000000, 0.000000000000000000, 1.000000000000000000 ) ) ;
#24551=VERTEX_POINT ( 'NONE', #96503 ) ;
#24552=CARTESIAN_POINT ( 'NONE',  ( -1.250000000000037970, 12.50000000000000000, 7.188010851410848723 ) ) ;
#24553=CONICAL_SURFACE ( 'NONE', #97700, 0.1000000000000002554, 0.003490658503988666988 ) ;
#24554=AXIS2_PLACEMENT_3D ( 'NONE', #59218, #3501, #51337 ) ;
#24555=FACE_OUTER_BOUND ( 'NONE', #31313, .T. ) ;
#24556=ORIENTED_EDGE ( 'NONE', *, *, #20023, .F. ) ;
#24557=ORIENTED_EDGE ( 'NONE', *, *, #164, .F. ) ;
#24558=EDGE_CURVE ( 'NONE', #5496, #93617, #124707, .T. ) ;
#24560=CARTESIAN_POINT ( 'NONE',  ( 9.599999999999914380, 12.50000000000000000, -4.265033745738164406 ) ) ;
#24561=DIRECTION ( 'NONE',  ( 0.000000000000000000, 0.000000000000000000, -1.000000000000000000 ) ) ;
#24564=CONICAL_SURFACE ( 'NONE', #116489, 0.09999999999999982514, 0.003490658503988666988 ) ;
#24565=VECTOR ( 'NONE', #102015, 1000.000000000000000 ) ;
#24566=VECTOR ( 'NONE', #53199, 1000.000000000000000 ) ;
#24567=DIRECTION ( 'NONE',  ( -0.000000000000000000, 1.000000000000000000, -0.000000000000000000 ) ) ;
#24568=LINE ( 'NONE', #57254, #17269 ) ;
#24569=AXIS2_PLACEMENT_3D ( 'NONE', #6836, #17970, #16662 ) ;
#24570=ORIENTED_EDGE ( 'NONE', *, *, #60264, .F. ) ;
#24571=FACE_OUTER_BOUND ( 'NONE', #115179, .T. ) ;
#24572=CONICAL_SURFACE ( 'NONE', #97723, 0.09999999999999982514, 0.003490658503988666988 ) ;
#24573=EDGE_CURVE ( 'NONE', #53445, #85857, #65410, .T. ) ;
#24574=ORIENTED_EDGE ( 'NONE', *, *, #80141, .T. ) ;
#24575=CARTESIAN_POINT ( 'NONE',  ( 4.999999999999933387, 2.500000000000000000, 4.922947341949748257 ) ) ;
#24576=DIRECTION ( 'NONE',  ( 0.000000000000000000, 1.000000000000000000, 0.000000000000000000 ) ) ;
#24577=DIRECTION ( 'NONE',  ( -4.274815082592931898E-19, -0.9999939076577903929, -0.003490651415223739937 ) ) ;
#24578=ORIENTED_EDGE ( 'NONE', *, *, #47233, .T. ) ;
#24579=EDGE_CURVE ( 'NONE', #31361, #33917, #52800, .T. ) ;
#24580=CIRCLE ( 'NONE', #114459, 0.06509327318403745899 ) ;
#24581=DIRECTION ( 'NONE',  ( -0.000000000000000000, -1.000000000000000000, -0.000000000000000000 ) ) ;
#24582=DIRECTION ( 'NONE',  ( 0.000000000000000000, 0.000000000000000000, 1.000000000000000000 ) ) ;
#24583=AXIS2_PLACEMENT_3D ( 'NONE', #92108, #62673, #24034 ) ;
#24584=EDGE_CURVE ( 'NONE', #76293, #70678, #50756, .T. ) ;
#24585=ADVANCED_FACE ( 'NONE', ( #105714 ), #27756, .T. ) ;
#24586=ADVANCED_FACE ( 'NONE', ( #6827 ), #115569, .T. ) ;
#24587=AXIS2_PLACEMENT_3D ( 'NONE', #35309, #96772, #126903 ) ;
#24588=EDGE_CURVE ( 'NONE', #75028, #110459, #73717, .T. ) ;
#24589=ORIENTED_EDGE ( 'NONE', *, *, #81077, .T. ) ;
#24590=AXIS2_PLACEMENT_3D ( 'NONE', #99310, #57451, #58740 ) ;
#24592=CONICAL_SURFACE ( 'NONE', #55888, 0.09999999999999999167, 0.003490658503988666988 ) ;
#24593=ORIENTED_EDGE ( 'NONE', *, *, #98876, .F. ) ;
#24594=ORIENTED_EDGE ( 'NONE', *, *, #127627, .T. ) ;
#24595=DIRECTION ( 'NONE',  ( 0.000000000000000000, 0.000000000000000000, 1.000000000000000000 ) ) ;
#24596=EDGE_CURVE ( 'NONE', #12708, #63537, #29827, .T. ) ;
#24598=CIRCLE ( 'NONE', #83196, 0.1000000000000000056 ) ;
#24599=ORIENTED_EDGE ( 'NONE', *, *, #63284, .T. ) ;
#24600=CARTESIAN_POINT ( 'NONE',  ( 3.749999999999944045, 2.500000000000000000, -2.757883832488654097 ) ) ;
#24601=CARTESIAN_POINT ( 'NONE',  ( -14.14999999999998614, 12.50000000000000000, 2.165063509461101265 ) ) ;
#24602=AXIS2_PLACEMENT_3D ( 'NONE', #12726, #120769, #111591 ) ;
#24603=CARTESIAN_POINT ( 'NONE',  ( 8.749999999999923617, 2.500000000000000000, 1.472243186433545459 ) ) ;
#24604=ORIENTED_EDGE ( 'NONE', *, *, #83070, .T. ) ;
#24605=ADVANCED_FACE ( 'NONE', ( #84778 ), #86710, .T. ) ;
#24606=CIRCLE ( 'NONE', #106181, 0.06509327318403745899 ) ;
#24607=FACE_BOUND ( 'NONE', #121572, .T. ) ;
#24608=EDGE_CURVE ( 'NONE', #46684, #99945, #56987, .T. ) ;
#24609=DIRECTION ( 'NONE',  ( -0.000000000000000000, 1.000000000000000000, -0.000000000000000000 ) ) ;
#24610=CARTESIAN_POINT ( 'NONE',  ( -5.600000000000020073, 2.500000000000000000, 0.3464101615137736845 ) ) ;
#24611=ORIENTED_EDGE ( 'NONE', *, *, #25468, .T. ) ;
#24612=CARTESIAN_POINT ( 'NONE',  ( 12.09999999999990550, 2.500000000000000000, -3.537306695894649966 ) ) ;
#24613=AXIS2_PLACEMENT_3D ( 'NONE', #87456, #89408, #69114 ) ;
#24614=EDGE_CURVE ( 'NONE', #59573, #11927, #106973, .T. ) ;
#24615=LINE ( 'NONE', #46180, #96919 ) ;
#24616=EDGE_CURVE ( 'NONE', #114539, #97064, #24568, .T. ) ;
#24617=EDGE_LOOP ( 'NONE', ( #103878, #78783 ) ) ;
#24618=AXIS2_PLACEMENT_3D ( 'NONE', #75401, #125162, #44672 ) ;
#24619=AXIS2_PLACEMENT_3D ( 'NONE', #115361, #87850, #65644 ) ;
#24620=VERTEX_POINT ( 'NONE', #7494 ) ;
#24621=ORIENTED_EDGE ( 'NONE', *, *, #123740, .F. ) ;
#24622=CARTESIAN_POINT ( 'NONE',  ( 5.849999999999931255, 2.500000000000000000, 2.957883832488649389 ) ) ;
#24623=DIRECTION ( 'NONE',  ( 0.000000000000000000, 1.000000000000000000, 0.000000000000000000 ) ) ;
#24624=CARTESIAN_POINT ( 'NONE',  ( -8.350000000000013856, 12.50000000000000000, -2.165063509461101710 ) ) ;
#24626=FACE_BOUND ( 'NONE', #30164, .T. ) ;
#24627=ORIENTED_EDGE ( 'NONE', *, *, #109900, .T. ) ;
#24629=LINE ( 'NONE', #124757, #107614 ) ;
#24630=CARTESIAN_POINT ( 'NONE',  ( 3.949999999999939782, 2.500000000000000000, 2.611473670974873151 ) ) ;
#24631=FACE_OUTER_BOUND ( 'NONE', #36603, .T. ) ;
#24632=DIRECTION ( 'NONE',  ( 0.000000000000000000, 1.000000000000000000, 0.000000000000000000 ) ) ;
#24633=DIRECTION ( 'NONE',  ( -0.000000000000000000, 1.000000000000000000, -0.000000000000000000 ) ) ;
#24634=DIRECTION ( 'NONE',  ( 0.000000000000000000, 1.000000000000000000, 0.000000000000000000 ) ) ;
#24635=DIRECTION ( 'NONE',  ( -4.274815082592931898E-19, -0.9999939076577903929, -0.003490651415223739937 ) ) ;
#24636=ORIENTED_EDGE ( 'NONE', *, *, #87502, .F. ) ;
#24637=ORIENTED_EDGE ( 'NONE', *, *, #40412, .F. ) ;
#24638=ORIENTED_EDGE ( 'NONE', *, *, #103761, .F. ) ;
#24639=ORIENTED_EDGE ( 'NONE', *, *, #84587, .T. ) ;
#24640=ORIENTED_EDGE ( 'NONE', *, *, #114393, .F. ) ;
#24641=FACE_OUTER_BOUND ( 'NONE', #52815, .T. ) ;
#24642=VECTOR ( 'NONE', #5645, 1000.000000000000000 ) ;
#24643=FACE_OUTER_BOUND ( 'NONE', #67835, .T. ) ;
#24644=ORIENTED_EDGE ( 'NONE', *, *, #124658, .T. ) ;
#24645=FACE_BOUND ( 'NONE', #33787, .T. ) ;
#24646=DIRECTION ( 'NONE',  ( 0.000000000000000000, 1.000000000000000000, 0.000000000000000000 ) ) ;
#24647=AXIS2_PLACEMENT_3D ( 'NONE', #102296, #61738, #11328 ) ;
#24648=EDGE_CURVE ( 'NONE', #4060, #114896, #94582, .T. ) ;
#24649=AXIS2_PLACEMENT_3D ( 'NONE', #100886, #121183, #72735 ) ;
#24651=EDGE_CURVE ( 'NONE', #83875, #40839, #48709, .T. ) ;
#24652=EDGE_LOOP ( 'NONE', ( #73723, #113327, #32998, #111449 ) ) ;
#24654=CARTESIAN_POINT ( 'NONE',  ( 1.899999999999951283, 12.50000000000000000, -4.611443907251939756 ) ) ;
#24655=CARTESIAN_POINT ( 'NONE',  ( -5.400000000000020783, 2.500000000000000000, 0.6928203230275494784 ) ) ;
#24656=EDGE_LOOP ( 'NONE', ( #7069, #128520, #10153, #100922 ) ) ;
#24657=CARTESIAN_POINT ( 'NONE',  ( -5.650000000000019895, 2.500000000000000000, 1.818653347947321475 ) ) ;
#24658=AXIS2_PLACEMENT_3D ( 'NONE', #92976, #42597, #72687 ) ;
#24659=EDGE_LOOP ( 'NONE', ( #50292, #32300, #71696, #12808 ) ) ;
#24660=AXIS2_PLACEMENT_3D ( 'NONE', #82503, #72036, #91661 ) ;
#24661=AXIS2_PLACEMENT_3D ( 'NONE', #92444, #49972, #89862 ) ;
#24662=EDGE_LOOP ( 'NONE', ( #96735, #17541 ) ) ;
#24663=EDGE_LOOP ( 'NONE', ( #80809, #18932, #64886, #119370 ) ) ;
#24664=DIRECTION ( 'NONE',  ( 0.000000000000000000, 0.000000000000000000, 1.000000000000000000 ) ) ;
#24665=FACE_OUTER_BOUND ( 'NONE', #60746, .T. ) ;
#24666=FACE_OUTER_BOUND ( 'NONE', #118865, .T. ) ;
#24667=ORIENTED_EDGE ( 'NONE', *, *, #26714, .F. ) ;
#24668=CARTESIAN_POINT ( 'NONE',  ( 13.54999999999989768, 12.50000000000000000, -2.511473670974877948 ) ) ;
#24669=CIRCLE ( 'NONE', #108284, 0.06509327318403745899 ) ;
#24670=CARTESIAN_POINT ( 'NONE',  ( 2.499999999999983569, 12.50000000000000000, 0.06509327318403515528 ) ) ;
#24671=CARTESIAN_POINT ( 'NONE',  ( 0.1999999999999571565, 12.50000000000000000, 3.983716857408420076 ) ) ;
#24672=PLANE ( 'NONE',  #24583 ) ;
#24673=DIRECTION ( 'NONE',  ( -0.000000000000000000, 1.000000000000000000, -0.000000000000000000 ) ) ;
#24674=EDGE_LOOP ( 'NONE', ( #111034, #20408 ) ) ;
#24675=CIRCLE ( 'NONE', #85298, 0.06509327318403745899 ) ;
#24676=CARTESIAN_POINT ( 'NONE',  ( -2.900000000000029221, 2.500000000000000000, -2.276824562219559311E-15 ) ) ;
#24677=ORIENTED_EDGE ( 'NONE', *, *, #6084, .F. ) ;
#24678=CARTESIAN_POINT ( 'NONE',  ( -14.39999999999998614, 2.500000000000000000, -0.3464101615137760715 ) ) ;
#24679=AXIS2_PLACEMENT_3D ( 'NONE', #42667, #76463, #83222 ) ;
#24681=ORIENTED_EDGE ( 'NONE', *, *, #80, .F. ) ;
#24682=DIRECTION ( 'NONE',  ( 0.000000000000000000, 0.000000000000000000, 1.000000000000000000 ) ) ;
#24684=FACE_OUTER_BOUND ( 'NONE', #81245, .T. ) ;
#24685=CARTESIAN_POINT ( 'NONE',  ( -11.25000000000000178, 12.50000000000000000, -1.472243186433546125 ) ) ;
#24686=LINE ( 'NONE', #77003, #105220 ) ;
#24687=DIRECTION ( 'NONE',  ( -0.000000000000000000, -1.000000000000000000, -0.000000000000000000 ) ) ;
#24688=CIRCLE ( 'NONE', #97829, 0.06509327318403745899 ) ;
#24689=ORIENTED_EDGE ( 'NONE', *, *, #104676, .F. ) ;
#24690=AXIS2_PLACEMENT_3D ( 'NONE', #90352, #89088, #80561 ) ;
#24691=ORIENTED_EDGE ( 'NONE', *, *, #86521, .T. ) ;
#24692=ADVANCED_FACE ( 'NONE', ( #30392 ), #111365, .T. ) ;
#24694=AXIS2_PLACEMENT_3D ( 'NONE', #83364, #24435, #55825 ) ;
#24695=CARTESIAN_POINT ( 'NONE',  ( -4.150000000000025224, 12.50000000000000000, 5.867463478539781896 ) ) ;
#24696=DIRECTION ( 'NONE',  ( 0.000000000000000000, 0.000000000000000000, 1.000000000000000000 ) ) ;
#24697=ORIENTED_EDGE ( 'NONE', *, *, #119429, .F. ) ;
#24698=EDGE_LOOP ( 'NONE', ( #110186, #118650 ) ) ;
#24699=DIRECTION ( 'NONE',  ( 0.000000000000000000, -0.000000000000000000, 1.000000000000000000 ) ) ;
#24700=AXIS2_PLACEMENT_3D ( 'NONE', #124482, #47213, #125125 ) ;
#24701=VERTEX_POINT ( 'NONE', #77526 ) ;
#24702=FACE_OUTER_BOUND ( 'NONE', #108157, .T. ) ;
#24703=DIRECTION ( 'NONE',  ( 0.000000000000000000, 0.000000000000000000, 1.000000000000000000 ) ) ;
#24704=VERTEX_POINT ( 'NONE', #10698 ) ;
#24705=DIRECTION ( 'NONE',  ( 0.000000000000000000, -0.000000000000000000, 1.000000000000000000 ) ) ;
#24706=DIRECTION ( 'NONE',  ( 0.000000000000000000, 0.000000000000000000, 1.000000000000000000 ) ) ;
#24707=LINE ( 'NONE', #6963, #5022 ) ;
#24708=EDGE_CURVE ( 'NONE', #55428, #2826, #4756, .T. ) ;
#24709=VECTOR ( 'NONE', #71466, 1000.000000000000000 ) ;
#24710=EDGE_CURVE ( 'NONE', #107893, #4124, #108907, .T. ) ;
#24711=CARTESIAN_POINT ( 'NONE',  ( 6.049999999999932321, 2.500000000000000000, 1.918653347947321564 ) ) ;
#24712=ORIENTED_EDGE ( 'NONE', *, *, #51328, .F. ) ;
#24713=CARTESIAN_POINT ( 'NONE',  ( -0.6000000000000383915, 2.500000000000000000, -4.676537180435977881 ) ) ;
#24715=CARTESIAN_POINT ( 'NONE',  ( 11.84999999999990372, 2.500000000000000000, 1.718653347947321386 ) ) ;
#24716=ORIENTED_EDGE ( 'NONE', *, *, #27200, .T. ) ;
#24717=ORIENTED_EDGE ( 'NONE', *, *, #9948, .T. ) ;
#24718=ADVANCED_FACE ( 'NONE', ( #127921 ), #75877, .T. ) ;
#24720=PLANE ( 'NONE',  #122233 ) ;
#24721=CARTESIAN_POINT ( 'NONE',  ( 3.349999999999945466, 2.500000000000000000, -2.857883832488653741 ) ) ;
#24722=DIRECTION ( 'NONE',  ( 0.000000000000000000, 0.000000000000000000, 1.000000000000000000 ) ) ;
#24723=DIRECTION ( 'NONE',  ( 0.000000000000000000, -0.9999939076577903929, 0.003490651415223739937 ) ) ;
#24724=CARTESIAN_POINT ( 'NONE',  ( -10.60000000000000320, 2.500000000000000000, -3.883716857408422207 ) ) ;
#24725=CARTESIAN_POINT ( 'NONE',  ( -14.19999999999998685, 2.500000000000000000, -0.1000000000000001166 ) ) ;
#24726=CARTESIAN_POINT ( 'NONE',  ( 11.64999999999990798, 12.50000000000000000, -1.472243186433550122 ) ) ;
#24727=FACE_OUTER_BOUND ( 'NONE', #51275, .T. ) ;
#24728=CARTESIAN_POINT ( 'NONE',  ( -9.550000000000007816, 12.50000000000000000, -6.495190528383297135 ) ) ;
#24729=EDGE_LOOP ( 'NONE', ( #43614, #15304, #2163, #89077 ) ) ;
#24730=ORIENTED_EDGE ( 'NONE', *, *, #93730, .T. ) ;
#24731=EDGE_LOOP ( 'NONE', ( #112021, #100565 ) ) ;
#24732=AXIS2_PLACEMENT_3D ( 'NONE', #12421, #69409, #92269 ) ;
#24733=AXIS2_PLACEMENT_3D ( 'NONE', #10361, #77800, #78484 ) ;
#24734=EDGE_LOOP ( 'NONE', ( #95651, #55399 ) ) ;
#24735=CARTESIAN_POINT ( 'NONE',  ( -14.14999999999998614, 2.500000000000000000, -2.857883832488651521 ) ) ;
#24736=DIRECTION ( 'NONE',  ( 0.000000000000000000, 1.000000000000000000, 0.000000000000000000 ) ) ;
#24737=FACE_OUTER_BOUND ( 'NONE', #21578, .T. ) ;
#24738=EDGE_LOOP ( 'NONE', ( #82328, #1885, #88731, #34845 ) ) ;
#24739=VECTOR ( 'NONE', #60301, 1000.000000000000000 ) ;
#24740=PLANE ( 'NONE',  #29921 ) ;
#24741=EDGE_CURVE ( 'NONE', #37904, #74337, #59177, .T. ) ;
#24742=CIRCLE ( 'NONE', #33160, 0.1000000000000002554 ) ;
#24743=FACE_OUTER_BOUND ( 'NONE', #64967, .T. ) ;
#24744=DIRECTION ( 'NONE',  ( 0.000000000000000000, 0.000000000000000000, 1.000000000000000000 ) ) ;
#24745=ORIENTED_EDGE ( 'NONE', *, *, #84572, .T. ) ;
#24747=DIRECTION ( 'NONE',  ( 0.000000000000000000, 0.000000000000000000, 1.000000000000000000 ) ) ;
#24748=AXIS2_PLACEMENT_3D ( 'NONE', #34617, #114430, #24780 ) ;
#24749=EDGE_CURVE ( 'NONE', #70878, #48804, #29720, .T. ) ;
#24750=FACE_OUTER_BOUND ( 'NONE', #20433, .T. ) ;
#24751=ORIENTED_EDGE ( 'NONE', *, *, #105190, .F. ) ;
#24752=CONICAL_SURFACE ( 'NONE', #118742, 0.1000000000000002554, 0.003490658503988666988 ) ;
#24753=VERTEX_POINT ( 'NONE', #90570 ) ;
#24754=ORIENTED_EDGE ( 'NONE', *, *, #30858, .T. ) ;
#24755=VERTEX_POINT ( 'NONE', #88645 ) ;
#24757=ADVANCED_FACE ( 'NONE', ( #69646 ), #37623, .T. ) ;
#24759=EDGE_CURVE ( 'NONE', #90702, #17926, #103072, .T. ) ;
#24760=ADVANCED_FACE ( 'NONE', ( #59861 ), #52992, .T. ) ;
#24761=CARTESIAN_POINT ( 'NONE',  ( -7.050000000000016698, 2.500000000000000000, -2.065063509461102065 ) ) ;
#24762=FACE_OUTER_BOUND ( 'NONE', #81524, .T. ) ;
#24763=DIRECTION ( 'NONE',  ( 0.000000000000000000, 0.000000000000000000, 1.000000000000000000 ) ) ;
#24765=VERTEX_POINT ( 'NONE', #107645 ) ;
#24766=EDGE_CURVE ( 'NONE', #102282, #108236, #8770, .T. ) ;
#24767=CARTESIAN_POINT ( 'NONE',  ( -7.100000000000013856, 2.500000000000000000, 4.922947341949748257 ) ) ;
#24768=ORIENTED_EDGE ( 'NONE', *, *, #56075, .T. ) ;
#24769=AXIS2_PLACEMENT_3D ( 'NONE', #122614, #50643, #40853 ) ;
#24770=DIRECTION ( 'NONE',  ( 0.000000000000000000, 0.000000000000000000, 1.000000000000000000 ) ) ;
#24771=FACE_OUTER_BOUND ( 'NONE', #77137, .T. ) ;
#24772=CARTESIAN_POINT ( 'NONE',  ( -14.79999999999998295, 2.500000000000000000, -0.3464101615137760715 ) ) ;
#24773=CARTESIAN_POINT ( 'NONE',  ( 17.17539648375908712, -2.541523116374657221, 5.507477068181874102 ) ) ;
#24774=EDGE_CURVE ( 'NONE', #113894, #111448, #80096, .T. ) ;
#24775=ORIENTED_EDGE ( 'NONE', *, *, #4004, .T. ) ;
#24776=CIRCLE ( 'NONE', #28982, 0.09999999999999999167 ) ;
#24777=EDGE_LOOP ( 'NONE', ( #41894, #116576, #78659, #50920 ) ) ;
#24778=VERTEX_POINT ( 'NONE', #40195 ) ;
#24779=CARTESIAN_POINT ( 'NONE',  ( 4.349999999999937472, 12.50000000000000000, 6.776507416713035248 ) ) ;
#24780=DIRECTION ( 'NONE',  ( 0.000000000000000000, 0.000000000000000000, 1.000000000000000000 ) ) ;
#24781=CARTESIAN_POINT ( 'NONE',  ( 7.099999999999927702, 2.500000000000000000, 5.022947341949748790 ) ) ;
#24782=FACE_BOUND ( 'NONE', #81804, .T. ) ;
#24783=CARTESIAN_POINT ( 'NONE',  ( -8.150000000000014566, 2.500000000000000000, -6.941600689897073906 ) ) ;
#24784=CARTESIAN_POINT ( 'NONE',  ( 7.899999999999924860, 2.500000000000000000, 3.637306695894644726 ) ) ;
#24785=CARTESIAN_POINT ( 'NONE',  ( -9.550000000000002487, 2.500000000000000000, 6.595190528383296780 ) ) ;
#24786=CIRCLE ( 'NONE', #12241, 0.06509327318403745899 ) ;
#24788=DIRECTION ( 'NONE',  ( 0.000000000000000000, 0.000000000000000000, 1.000000000000000000 ) ) ;
#24789=VECTOR ( 'NONE', #6586, 1000.000000000000000 ) ;
#24790=DIRECTION ( 'NONE',  ( 0.000000000000000000, 0.000000000000000000, -1.000000000000000000 ) ) ;
#24791=VERTEX_POINT ( 'NONE', #110222 ) ;
#24792=CARTESIAN_POINT ( 'NONE',  ( -1.850000000000033396, 2.500000000000000000, -6.148780366869526226 ) ) ;
#24793=ORIENTED_EDGE ( 'NONE', *, *, #10662, .T. ) ;
#24795=EDGE_LOOP ( 'NONE', ( #15501, #57796, #76443, #1240 ) ) ;
#24796=ORIENTED_EDGE ( 'NONE', *, *, #22410, .T. ) ;
#24797=CONICAL_SURFACE ( 'NONE', #18527, 0.1000000000000002554, 0.003490658503988666988 ) ;
#24798=FACE_OUTER_BOUND ( 'NONE', #6584, .T. ) ;
#24799=FACE_BOUND ( 'NONE', #67251, .T. ) ;
#24800=DIRECTION ( 'NONE',  ( 0.000000000000000000, 0.000000000000000000, -1.000000000000000000 ) ) ;
#24802=CIRCLE ( 'NONE', #97954, 0.06509327318403745899 ) ;
#24803=ADVANCED_FACE ( 'NONE', ( #20555 ), #52907, .T. ) ;
#24804=ORIENTED_EDGE ( 'NONE', *, *, #1118, .T. ) ;
#24805=CARTESIAN_POINT ( 'NONE',  ( 21.15177371151419194, 2.593223176056360657, 4.151029080743467325 ) ) ;
#24806=FACE_OUTER_BOUND ( 'NONE', #14436, .T. ) ;
#24807=EDGE_LOOP ( 'NONE', ( #51738, #103142 ) ) ;
#24808=DIRECTION ( 'NONE',  ( 0.000000000000000000, 1.000000000000000000, 0.000000000000000000 ) ) ;
#24809=CARTESIAN_POINT ( 'NONE',  ( 3.349999999999945466, 2.500000000000000000, -7.188010851410854052 ) ) ;
#24810=EDGE_CURVE ( 'NONE', #107604, #53683, #101016, .T. ) ;
#24811=ORIENTED_EDGE ( 'NONE', *, *, #116909, .T. ) ;
#24812=CIRCLE ( 'NONE', #97967, 0.1000000000000002554 ) ;
#24813=DIRECTION ( 'NONE',  ( 0.000000000000000000, 0.000000000000000000, 1.000000000000000000 ) ) ;
#24814=PLANE ( 'NONE',  #51739 ) ;
#24815=ORIENTED_EDGE ( 'NONE', *, *, #100647, .F. ) ;
#24816=CIRCLE ( 'NONE', #33250, 0.09999999999999982514 ) ;
#24817=LINE ( 'NONE', #36593, #126224 ) ;
#24818=AXIS2_PLACEMENT_3D ( 'NONE', #65437, #123698, #64796 ) ;
#24819=CARTESIAN_POINT ( 'NONE',  ( -12.49999999999999467, 2.500000000000000000, -3.637306695894647390 ) ) ;
#24820=AXIS2_PLACEMENT_3D ( 'NONE', #22782, #91498, #1820 ) ;
#24821=DIRECTION ( 'NONE',  ( 0.000000000000000000, -0.9999939076577903929, 0.003490651415223739937 ) ) ;
#24822=EDGE_LOOP ( 'NONE', ( #121322, #46581 ) ) ;
#24823=ORIENTED_EDGE ( 'NONE', *, *, #116909, .F. ) ;
#24824=CARTESIAN_POINT ( 'NONE',  ( 11.89999999999990443, 12.50000000000000000, -0.4115034346978156399 ) ) ;
#24825=CIRCLE ( 'NONE', #3887, 0.06509327318403745899 ) ;
#24826=ORIENTED_EDGE ( 'NONE', *, *, #74779, .F. ) ;
#24827=DIRECTION ( 'NONE',  ( 0.000000000000000000, 0.000000000000000000, 1.000000000000000000 ) ) ;
#24828=PLANE ( 'NONE',  #99650 ) ;
#24829=AXIS2_PLACEMENT_3D ( 'NONE', #51604, #41793, #81060 ) ;
#24830=CIRCLE ( 'NONE', #100147, 0.1000000000000002554 ) ;
#24831=EDGE_LOOP ( 'NONE', ( #18031, #101729, #52173, #2169 ) ) ;
#24832=DIRECTION ( 'NONE',  ( -0.000000000000000000, 1.000000000000000000, -0.000000000000000000 ) ) ;
#24833=CARTESIAN_POINT ( 'NONE',  ( 7.899999999999924860, 2.500000000000000000, 3.637306695894644726 ) ) ;
#24834=CARTESIAN_POINT ( 'NONE',  ( 2.899999999999945732, 2.500000000000000000, -2.385244779468109755E-15 ) ) ;
#24835=CARTESIAN_POINT ( 'NONE',  ( 5.199999999999933564, 12.50000000000000000, 0.4115034346978109769 ) ) ;
#24836=DIRECTION ( 'NONE',  ( -4.274815082592931898E-19, -0.9999939076577903929, -0.003490651415223739937 ) ) ;
#24837=VECTOR ( 'NONE', #27186, 1000.000000000000000 ) ;
#24838=VERTEX_POINT ( 'NONE', #61782 ) ;
#24839=AXIS2_PLACEMENT_3D ( 'NONE', #77845, #109903, #48397 ) ;
#24840=EDGE_CURVE ( 'NONE', #58497, #119313, #109427, .T. ) ;
#24841=ORIENTED_EDGE ( 'NONE', *, *, #40313, .F. ) ;
#24842=DIRECTION ( 'NONE',  ( -0.000000000000000000, -1.000000000000000000, -0.000000000000000000 ) ) ;
#24843=DIRECTION ( 'NONE',  ( -0.000000000000000000, -1.000000000000000000, -0.000000000000000000 ) ) ;
#24844=CARTESIAN_POINT ( 'NONE',  ( -11.05000000000000249, 12.50000000000000000, -6.148780366869522673 ) ) ;
#24845=EDGE_LOOP ( 'NONE', ( #98785, #70382, #126492, #78589 ) ) ;
#24846=ORIENTED_EDGE ( 'NONE', *, *, #82123, .F. ) ;
#24848=DIRECTION ( 'NONE',  ( -0.000000000000000000, 1.000000000000000000, -0.000000000000000000 ) ) ;
#24849=CONICAL_SURFACE ( 'NONE', #127266, 0.1000000000000002554, 0.003490658503988666988 ) ;
#24850=DIRECTION ( 'NONE',  ( -4.274815082592931898E-19, -0.9999939076577903929, -0.003490651415223739937 ) ) ;
#24851=EDGE_CURVE ( 'NONE', #102186, #73740, #11370, .T. ) ;
#24852=DIRECTION ( 'NONE',  ( 0.000000000000000000, 0.000000000000000000, -1.000000000000000000 ) ) ;
#24854=DIRECTION ( 'NONE',  ( -0.000000000000000000, -1.000000000000000000, -0.000000000000000000 ) ) ;
#24855=DIRECTION ( 'NONE',  ( 0.000000000000000000, 0.000000000000000000, 1.000000000000000000 ) ) ;
#24856=LINE ( 'NONE', #96163, #123858 ) ;
#24857=DIRECTION ( 'NONE',  ( 0.000000000000000000, -0.000000000000000000, 1.000000000000000000 ) ) ;
#24858=CARTESIAN_POINT ( 'NONE',  ( 2.099999999999948574, 12.50000000000000000, 4.330127018922196314 ) ) ;
#24859=EDGE_CURVE ( 'NONE', #128359, #41239, #115674, .T. ) ;
#24860=EDGE_CURVE ( 'NONE', #64737, #11527, #121321, .T. ) ;
#24861=FACE_OUTER_BOUND ( 'NONE', #88022, .T. ) ;
#24862=VERTEX_POINT ( 'NONE', #43436 ) ;
#24863=CONICAL_SURFACE ( 'NONE', #28790, 0.1000000000000000472, 0.003490658503988666988 ) ;
#24864=EDGE_CURVE ( 'NONE', #113778, #52806, #11111, .T. ) ;
#24865=DIRECTION ( 'NONE',  ( 0.000000000000000000, -0.9999939076577903929, 0.003490651415223739937 ) ) ;
#24866=ORIENTED_EDGE ( 'NONE', *, *, #103669, .T. ) ;
#24867=ORIENTED_EDGE ( 'NONE', *, *, #83503, .T. ) ;
#24868=EDGE_CURVE ( 'NONE', #80261, #22096, #90548, .T. ) ;
#24869=DIRECTION ( 'NONE',  ( 0.000000000000000000, 1.000000000000000000, 0.000000000000000000 ) ) ;
#24870=CARTESIAN_POINT ( 'NONE',  ( -6.850000000000013856, 12.50000000000000000, 6.906693963081109722 ) ) ;
#24872=DIRECTION ( 'NONE',  ( 0.000000000000000000, 0.000000000000000000, 1.000000000000000000 ) ) ;
#24873=CARTESIAN_POINT ( 'NONE',  ( 5.649999999999934630, 12.50000000000000000, -1.883746621131363375 ) ) ;
#24874=AXIS2_PLACEMENT_3D ( 'NONE', #126347, #56930, #96870 ) ;
#24875=LINE ( 'NONE', #54969, #15108 ) ;
#24876=CARTESIAN_POINT ( 'NONE',  ( -6.450000000000019718, 2.500000000000000000, -6.048780366869526581 ) ) ;
#24877=DIRECTION ( 'NONE',  ( 0.000000000000000000, 1.000000000000000000, 0.000000000000000000 ) ) ;
#24878=EDGE_LOOP ( 'NONE', ( #116786, #47663 ) ) ;
#24879=FACE_OUTER_BOUND ( 'NONE', #67007, .T. ) ;
#24880=AXIS2_PLACEMENT_3D ( 'NONE', #14032, #53344, #53979 ) ;
#24881=DIRECTION ( 'NONE',  ( -4.274815082592931898E-19, -0.9999939076577903929, -0.003490651415223739937 ) ) ;
#24882=VERTEX_POINT ( 'NONE', #51955 ) ;
#24883=ORIENTED_EDGE ( 'NONE', *, *, #26654, .T. ) ;
#24884=AXIS2_PLACEMENT_3D ( 'NONE', #95, #59698, #99603 ) ;
#24885=ORIENTED_EDGE ( 'NONE', *, *, #114279, .T. ) ;
#24886=CIRCLE ( 'NONE', #108502, 0.1000000000000002554 ) ;
#24887=EDGE_LOOP ( 'NONE', ( #116915, #73786, #25533, #129098 ) ) ;
#24889=CARTESIAN_POINT ( 'NONE',  ( 8.549999999999918998, 2.500000000000000000, 6.841600689897072485 ) ) ;
#24892=DIRECTION ( 'NONE',  ( 0.000000000000000000, -0.000000000000000000, 1.000000000000000000 ) ) ;
#24893=DIRECTION ( 'NONE',  ( 0.000000000000000000, 0.000000000000000000, -1.000000000000000000 ) ) ;
#24894=ORIENTED_EDGE ( 'NONE', *, *, #50899, .T. ) ;
#24895=FACE_OUTER_BOUND ( 'NONE', #74620, .T. ) ;
#24896=CARTESIAN_POINT ( 'NONE',  ( -6.250000000000017764, 2.500000000000000000, 7.188010851410848723 ) ) ;
#24897=EDGE_CURVE ( 'NONE', #80982, #48968, #102845, .T. ) ;
#24898=CARTESIAN_POINT ( 'NONE',  ( 7.899999999999924860, 2.500000000000000000, 5.022947341949748790 ) ) ;
#24899=ORIENTED_EDGE ( 'NONE', *, *, #25916, .T. ) ;
#24900=ORIENTED_EDGE ( 'NONE', *, *, #69043, .F. ) ;
#24901=ORIENTED_EDGE ( 'NONE', *, *, #106160, .T. ) ;
#24902=EDGE_CURVE ( 'NONE', #85816, #108779, #31660, .T. ) ;
#24903=AXIS2_PLACEMENT_3D ( 'NONE', #91945, #81483, #103040 ) ;
#24904=PLANE ( 'NONE',  #21593 ) ;
#24905=ADVANCED_FACE ( 'NONE', ( #122622 ), #111477, .T. ) ;
#24906=EDGE_CURVE ( 'NONE', #108234, #91772, #78031, .T. ) ;
#24907=ADVANCED_FACE ( 'NONE', ( #12645 ), #73826, .T. ) ;
#24908=LINE ( 'NONE', #8314, #15355 ) ;
#24909=DIRECTION ( 'NONE',  ( 0.000000000000000000, -0.000000000000000000, 1.000000000000000000 ) ) ;
#24910=AXIS2_PLACEMENT_3D ( 'NONE', #101380, #63385, #92184 ) ;
#24911=CONICAL_SURFACE ( 'NONE', #10244, 0.1000000000000000056, 0.003490658503988666988 ) ;
#24912=ADVANCED_FACE ( 'NONE', ( #92501 ), #94752, .T. ) ;
#24913=EDGE_LOOP ( 'NONE', ( #4429, #129596 ) ) ;
#24914=DIRECTION ( 'NONE',  ( 0.000000000000000000, 1.000000000000000000, 0.000000000000000000 ) ) ;
#24915=DIRECTION ( 'NONE',  ( 0.000000000000000000, 0.000000000000000000, -1.000000000000000000 ) ) ;
#24916=DIRECTION ( 'NONE',  ( 0.000000000000000000, -0.9999939076577903929, 0.003490651415223739937 ) ) ;
#24917=DIRECTION ( 'NONE',  ( -4.274815082592931898E-19, -0.9999939076577903929, -0.003490651415223739937 ) ) ;
#24918=DIRECTION ( 'NONE',  ( -0.000000000000000000, -1.000000000000000000, -0.000000000000000000 ) ) ;
#24919=CONICAL_SURFACE ( 'NONE', #129413, 0.1000000000000002554, 0.003490658503988666988 ) ;
#24920=AXIS2_PLACEMENT_3D ( 'NONE', #26005, #67170, #126122 ) ;
#24921=EDGE_CURVE ( 'NONE', #99497, #25372, #98961, .T. ) ;
#24922=ORIENTED_EDGE ( 'NONE', *, *, #99659, .T. ) ;
#24923=CONICAL_SURFACE ( 'NONE', #52121, 0.1000000000000000472, 0.003490658503988666988 ) ;
#24924=EDGE_CURVE ( 'NONE', #51310, #63382, #41507, .T. ) ;
#24925=CARTESIAN_POINT ( 'NONE',  ( -4.200000000000029488, 2.500000000000000000, -4.230127018922201998 ) ) ;
#24926=ORIENTED_EDGE ( 'NONE', *, *, #877, .T. ) ;
#24927=ORIENTED_EDGE ( 'NONE', *, *, #124751, .F. ) ;
#24928=DIRECTION ( 'NONE',  ( 0.000000000000000000, 1.000000000000000000, 0.000000000000000000 ) ) ;
#24929=FACE_BOUND ( 'NONE', #26755, .T. ) ;
#24930=VECTOR ( 'NONE', #55847, 1000.000000000000000 ) ;
#24931=DIRECTION ( 'NONE',  ( 0.000000000000000000, 1.000000000000000000, 0.000000000000000000 ) ) ;
#24932=CARTESIAN_POINT ( 'NONE',  ( 0.7999999999999548583, 2.500000000000000000, 4.330127018922196314 ) ) ;
#24933=CARTESIAN_POINT ( 'NONE',  ( -5.200000000000025935, 2.500000000000000000, -4.083716857408426826 ) ) ;
#24934=ORIENTED_EDGE ( 'NONE', *, *, #45714, .F. ) ;
#24935=EDGE_LOOP ( 'NONE', ( #2842, #69067, #52546, #46170 ) ) ;
#24936=FACE_OUTER_BOUND ( 'NONE', #76370, .T. ) ;
#24937=LINE ( 'NONE', #76616, #28064 ) ;
#24938=DIRECTION ( 'NONE',  ( 0.000000000000000000, 0.000000000000000000, 1.000000000000000000 ) ) ;
#24939=DIRECTION ( 'NONE',  ( -0.000000000000000000, 1.000000000000000000, -0.000000000000000000 ) ) ;
#24940=EDGE_LOOP ( 'NONE', ( #18182, #47348 ) ) ;
#24941=CARTESIAN_POINT ( 'NONE',  ( -5.850000000000021849, 2.500000000000000000, -2.857883832488653741 ) ) ;
#24942=LINE ( 'NONE', #4626, #114356 ) ;
#24943=CONICAL_SURFACE ( 'NONE', #100164, 0.09999999999999982514, 0.003490658503988666988 ) ;
#24944=ORIENTED_EDGE ( 'NONE', *, *, #93468, .F. ) ;
#24945=DIRECTION ( 'NONE',  ( 0.000000000000000000, 0.000000000000000000, -1.000000000000000000 ) ) ;
#24946=ORIENTED_EDGE ( 'NONE', *, *, #122494, .F. ) ;
#24947=FACE_BOUND ( 'NONE', #55866, .T. ) ;
#24948=CARTESIAN_POINT ( 'NONE',  ( -10.40000000000000213, 12.50000000000000000, 0.6928203230275494784 ) ) ;
#24949=ORIENTED_EDGE ( 'NONE', *, *, #11331, .F. ) ;
#24950=FACE_OUTER_BOUND ( 'NONE', #22004, .T. ) ;
#24951=DIRECTION ( 'NONE',  ( -0.000000000000000000, -1.000000000000000000, -0.000000000000000000 ) ) ;
#24952=EDGE_LOOP ( 'NONE', ( #120724, #68847, #69875, #91408 ) ) ;
#24953=ORIENTED_EDGE ( 'NONE', *, *, #48535, .F. ) ;
#24955=CONICAL_SURFACE ( 'NONE', #18692, 0.1000000000000000056, 0.003490658503988666988 ) ;
#24956=DIRECTION ( 'NONE',  ( -0.000000000000000000, 1.000000000000000000, -0.000000000000000000 ) ) ;
#24957=DIRECTION ( 'NONE',  ( -0.000000000000000000, 1.000000000000000000, -0.000000000000000000 ) ) ;
#24958=ADVANCED_FACE ( 'NONE', ( #93221 ), #29922, .T. ) ;
#24959=DIRECTION ( 'NONE',  ( -0.000000000000000000, 1.000000000000000000, -0.000000000000000000 ) ) ;
#24960=CARTESIAN_POINT ( 'NONE',  ( 4.999999999999936939, 2.500000000000000000, -0.7928203230275542301 ) ) ;
#24961=CARTESIAN_POINT ( 'NONE',  ( 1.249999999999953815, 12.50000000000000000, -2.922977105672691422 ) ) ;
#24962=DIRECTION ( 'NONE',  ( 0.000000000000000000, 0.000000000000000000, 1.000000000000000000 ) ) ;
#24963=VECTOR ( 'NONE', #84402, 1000.000000000000000 ) ;
#24964=ORIENTED_EDGE ( 'NONE', *, *, #76440, .T. ) ;
#24965=ORIENTED_EDGE ( 'NONE', *, *, #14966, .F. ) ;
#24966=DIRECTION ( 'NONE',  ( 0.000000000000000000, 0.000000000000000000, -1.000000000000000000 ) ) ;
#24967=AXIS2_PLACEMENT_3D ( 'NONE', #73340, #36509, #59379 ) ;
#24968=CONICAL_SURFACE ( 'NONE', #22928, 0.1000000000000000472, 0.003490658503988666988 ) ;
#24969=PLANE ( 'NONE',  #95686 ) ;
#24970=CARTESIAN_POINT ( 'NONE',  ( -6.450000000000016165, 2.500000000000000000, 2.611473670974873151 ) ) ;
#24971=LINE ( 'NONE', #83263, #53244 ) ;
#24973=ORIENTED_EDGE ( 'NONE', *, *, #64221, .F. ) ;
#24974=VERTEX_POINT ( 'NONE', #82100 ) ;
#24975=FACE_BOUND ( 'NONE', #20046, .T. ) ;
#24977=CARTESIAN_POINT ( 'NONE',  ( -0.6500000000000389910, 2.500000000000000000, -6.148780366869526226 ) ) ;
#24978=DIRECTION ( 'NONE',  ( 0.000000000000000000, 0.000000000000000000, 1.000000000000000000 ) ) ;
#24979=ORIENTED_EDGE ( 'NONE', *, *, #36333, .F. ) ;
#24980=DIRECTION ( 'NONE',  ( -0.000000000000000000, -1.000000000000000000, -0.000000000000000000 ) ) ;
#24981=CONICAL_SURFACE ( 'NONE', #45924, 0.1000000000000002554, 0.003490658503988666988 ) ;
#24982=AXIS2_PLACEMENT_3D ( 'NONE', #118130, #28476, #40727 ) ;
#24983=DIRECTION ( 'NONE',  ( 0.000000000000000000, 0.000000000000000000, 1.000000000000000000 ) ) ;
#24984=DIRECTION ( 'NONE',  ( 0.000000000000000000, 0.000000000000000000, -1.000000000000000000 ) ) ;
#24985=DIRECTION ( 'NONE',  ( 0.000000000000000000, 1.000000000000000000, 0.000000000000000000 ) ) ;
#24986=DIRECTION ( 'NONE',  ( 0.000000000000000000, 0.000000000000000000, -1.000000000000000000 ) ) ;
#24987=FACE_OUTER_BOUND ( 'NONE', #44055, .T. ) ;
#24988=DIRECTION ( 'NONE',  ( 0.000000000000000000, 1.000000000000000000, 0.000000000000000000 ) ) ;
#24989=DIRECTION ( 'NONE',  ( 0.000000000000000000, 1.000000000000000000, 0.000000000000000000 ) ) ;
#24990=CARTESIAN_POINT ( 'NONE',  ( 4.999999999999938716, 2.500000000000000000, -5.122947341949753763 ) ) ;
#24991=VERTEX_POINT ( 'NONE', #82765 ) ;
#24992=ORIENTED_EDGE ( 'NONE', *, *, #37157, .F. ) ;
#24993=ORIENTED_EDGE ( 'NONE', *, *, #112921, .T. ) ;
#24994=CARTESIAN_POINT ( 'NONE',  ( 14.59999999999989484, 12.50000000000000000, 0.6928203230275494784 ) ) ;
#24995=ORIENTED_EDGE ( 'NONE', *, *, #16988, .F. ) ;
#24996=DIRECTION ( 'NONE',  ( 0.000000000000000000, 0.000000000000000000, -1.000000000000000000 ) ) ;
#24997=CIRCLE ( 'NONE', #98145, 0.09999999999999982514 ) ;
#24998=VERTEX_POINT ( 'NONE', #52633 ) ;
#24999=ORIENTED_EDGE ( 'NONE', *, *, #74726, .F. ) ;
#25000=ORIENTED_EDGE ( 'NONE', *, *, #110957, .F. ) ;
#25001=DIRECTION ( 'NONE',  ( 0.000000000000000000, 0.000000000000000000, 1.000000000000000000 ) ) ;
#25002=AXIS2_PLACEMENT_3D ( 'NONE', #73519, #122636, #93820 ) ;
#25003=EDGE_CURVE ( 'NONE', #97516, #29211, #55044, .T. ) ;
#25004=CIRCLE ( 'NONE', #62671, 0.06509327318403745899 ) ;
#25005=DIRECTION ( 'NONE',  ( 0.000000000000000000, 0.000000000000000000, -1.000000000000000000 ) ) ;
#25006=DIRECTION ( 'NONE',  ( 0.000000000000000000, 0.000000000000000000, 1.000000000000000000 ) ) ;
#25007=DIRECTION ( 'NONE',  ( 0.000000000000000000, 0.000000000000000000, 1.000000000000000000 ) ) ;
#25008=EDGE_CURVE ( 'NONE', #94668, #84709, #34128, .T. ) ;
#25009=ORIENTED_EDGE ( 'NONE', *, *, #24040, .T. ) ;
#25010=EDGE_CURVE ( 'NONE', #28470, #22443, #74218, .T. ) ;
#25011=AXIS2_PLACEMENT_3D ( 'NONE', #56436, #106201, #17127 ) ;
#25012=VECTOR ( 'NONE', #111649, 1000.000000000000000 ) ;
#25013=CARTESIAN_POINT ( 'NONE',  ( -11.64999999999999858, 12.50000000000000000, -1.537336459617583584 ) ) ;
#25014=CIRCLE ( 'NONE', #106569, 0.06509327318403745899 ) ;
#25015=EDGE_LOOP ( 'NONE', ( #112542, #48371 ) ) ;
#25016=VECTOR ( 'NONE', #14995, 1000.000000000000000 ) ;
#25017=ORIENTED_EDGE ( 'NONE', *, *, #104987, .F. ) ;
#25018=ORIENTED_EDGE ( 'NONE', *, *, #101397, .T. ) ;
#25019=EDGE_CURVE ( 'NONE', #77356, #50837, #63370, .T. ) ;
#25020=CARTESIAN_POINT ( 'NONE',  ( -4.400000000000025224, 2.500000000000000000, -0.4464101615137783252 ) ) ;
#25021=ADVANCED_FACE ( 'NONE', ( #4163 ), #96798, .T. ) ;
#25022=EDGE_CURVE ( 'NONE', #21324, #18873, #40394, .T. ) ;
#25023=ORIENTED_EDGE ( 'NONE', *, *, #89569, .F. ) ;
#25024=ORIENTED_EDGE ( 'NONE', *, *, #64746, .T. ) ;
#25025=EDGE_CURVE ( 'NONE', #67610, #29442, #2818, .T. ) ;
#25026=VERTEX_POINT ( 'NONE', #112857 ) ;
#25027=VECTOR ( 'NONE', #100920, 1000.000000000000000 ) ;
#25028=DIRECTION ( 'NONE',  ( 0.000000000000000000, -0.000000000000000000, 1.000000000000000000 ) ) ;
#25030=DIRECTION ( 'NONE',  ( 0.000000000000000000, 1.000000000000000000, 0.000000000000000000 ) ) ;
#25031=DIRECTION ( 'NONE',  ( 0.000000000000000000, 1.000000000000000000, 0.000000000000000000 ) ) ;
#25032=DIRECTION ( 'NONE',  ( 0.000000000000000000, 0.000000000000000000, 1.000000000000000000 ) ) ;
#25033=DIRECTION ( 'NONE',  ( 0.000000000000000000, 1.000000000000000000, 0.000000000000000000 ) ) ;
#25034=VERTEX_POINT ( 'NONE', #103020 ) ;
#25035=EDGE_CURVE ( 'NONE', #36406, #90496, #75968, .T. ) ;
#25036=CARTESIAN_POINT ( 'NONE',  ( 13.34999999999990017, 2.500000000000000000, 1.472243186433545459 ) ) ;
#25037=CONICAL_SURFACE ( 'NONE', #64822, 0.09999999999999982514, 0.003490658503988666988 ) ;
#25038=VERTEX_POINT ( 'NONE', #83403 ) ;
#25039=FACE_OUTER_BOUND ( 'NONE', #37704, .T. ) ;
#25040=EDGE_LOOP ( 'NONE', ( #109205, #73944 ) ) ;
#25041=DIRECTION ( 'NONE',  ( -0.000000000000000000, 1.000000000000000000, -0.000000000000000000 ) ) ;
#25042=AXIS2_PLACEMENT_3D ( 'NONE', #81362, #28390, #34194 ) ;
#25044=VERTEX_POINT ( 'NONE', #52008 ) ;
#25045=DIRECTION ( 'NONE',  ( 0.000000000000000000, 1.000000000000000000, 0.000000000000000000 ) ) ;
#25046=LINE ( 'NONE', #104873, #44339 ) ;
#25047=DIRECTION ( 'NONE',  ( 0.000000000000000000, 0.000000000000000000, -1.000000000000000000 ) ) ;
#25048=DIRECTION ( 'NONE',  ( 0.000000000000000000, 0.000000000000000000, -1.000000000000000000 ) ) ;
#25049=ORIENTED_EDGE ( 'NONE', *, *, #28597, .T. ) ;
#25050=DIRECTION ( 'NONE',  ( 0.000000000000000000, 1.000000000000000000, 0.000000000000000000 ) ) ;
#25051=DIRECTION ( 'NONE',  ( -4.274815082592931898E-19, -0.9999939076577903929, -0.003490651415223739937 ) ) ;
#25052=DIRECTION ( 'NONE',  ( 0.000000000000000000, 1.000000000000000000, 0.000000000000000000 ) ) ;
#25053=DIRECTION ( 'NONE',  ( 0.000000000000000000, 0.000000000000000000, 1.000000000000000000 ) ) ;
#25054=DIRECTION ( 'NONE',  ( 0.000000000000000000, 0.000000000000000000, 1.000000000000000000 ) ) ;
#25055=ORIENTED_EDGE ( 'NONE', *, *, #36993, .T. ) ;
#25056=B_SPLINE_CURVE_WITH_KNOTS ( 'NONE', 3,
 ( #78797, #59815, #99716, #30992, #10647, #70893 ),
 .UNSPECIFIED., .F., .F.,
 ( 4, 2, 4 ),
 ( 0.000000000000000000, 0.5000000000000000000, 1.000000000000000000 ),
 .UNSPECIFIED. ) ;
#25057=EDGE_LOOP ( 'NONE', ( #119212, #46144, #47432, #51263 ) ) ;
#25058=EDGE_CURVE ( 'NONE', #60727, #7453, #42182, .T. ) ;
#25059=AXIS2_PLACEMENT_3D ( 'NONE', #57534, #99394, #8410 ) ;
#25060=EDGE_CURVE ( 'NONE', #16149, #31481, #69715, .T. ) ;
#25061=EDGE_LOOP ( 'NONE', ( #124617, #27477, #76506, #47568 ) ) ;
#25062=CARTESIAN_POINT ( 'NONE',  ( 10.84999999999990905, 12.50000000000000000, 2.230156782645134950 ) ) ;
#25063=DIRECTION ( 'NONE',  ( 0.000000000000000000, 0.000000000000000000, 1.000000000000000000 ) ) ;
#25064=ADVANCED_FACE ( 'NONE', ( #24472 ), #11425, .T. ) ;
#25065=CIRCLE ( 'NONE', #10392, 0.06509327318403745899 ) ;
#25067=DIRECTION ( 'NONE',  ( -4.274815082592931898E-19, -0.9999939076577903929, -0.003490651415223739937 ) ) ;
#25068=PLANE ( 'NONE',  #86261 ) ;
#25069=EDGE_CURVE ( 'NONE', #80728, #50779, #113485, .T. ) ;
#25070=DIRECTION ( 'NONE',  ( 0.000000000000000000, 0.000000000000000000, 1.000000000000000000 ) ) ;
#25071=CARTESIAN_POINT ( 'NONE',  ( 7.899999999999924860, 2.500000000000000000, 4.330127018922196314 ) ) ;
#25072=ORIENTED_EDGE ( 'NONE', *, *, #81032, .T. ) ;
#25073=EDGE_CURVE ( 'NONE', #103182, #85304, #55148, .T. ) ;
#25074=AXIS2_PLACEMENT_3D ( 'NONE', #112150, #44702, #23775 ) ;
#25075=CONICAL_SURFACE ( 'NONE', #8338, 0.1000000000000000472, 0.003490658503988666988 ) ;
#25076=ADVANCED_FACE ( 'NONE', ( #53301 ), #59371, .T. ) ;
#25077=EDGE_CURVE ( 'NONE', #107141, #53057, #73915, .T. ) ;
#25078=DIRECTION ( 'NONE',  ( -0.000000000000000000, 1.000000000000000000, -0.000000000000000000 ) ) ;
#25080=ORIENTED_EDGE ( 'NONE', *, *, #36355, .T. ) ;
#25081=EDGE_CURVE ( 'NONE', #41461, #66584, #80185, .T. ) ;
#25082=LINE ( 'NONE', #104907, #124234 ) ;
#25083=ORIENTED_EDGE ( 'NONE', *, *, #4301, .T. ) ;
#25084=CARTESIAN_POINT ( 'NONE',  ( 10.64999999999991331, 12.50000000000000000, -1.818653347947325916 ) ) ;
#25085=ORIENTED_EDGE ( 'NONE', *, *, #46155, .T. ) ;
#25086=FACE_OUTER_BOUND ( 'NONE', #4961, .T. ) ;
#25087=CARTESIAN_POINT ( 'NONE',  ( -9.350000000000006750, 12.50000000000000000, -2.511473670974877948 ) ) ;
#25088=DIRECTION ( 'NONE',  ( -0.000000000000000000, -1.000000000000000000, -0.000000000000000000 ) ) ;
#25089=ORIENTED_EDGE ( 'NONE', *, *, #63262, .F. ) ;
#25090=AXIS2_PLACEMENT_3D ( 'NONE', #3919, #83772, #113886 ) ;
#25091=CARTESIAN_POINT ( 'NONE',  ( 14.34999999999989306, 12.50000000000000000, -1.883746621131363597 ) ) ;
#25092=AXIS2_PLACEMENT_3D ( 'NONE', #86640, #37556, #7425 ) ;
#25093=CARTESIAN_POINT ( 'NONE',  ( 12.29999999999990123, 2.500000000000000000, 0.4464101615137735513 ) ) ;
#25094=ORIENTED_EDGE ( 'NONE', *, *, #111949, .F. ) ;
#25095=AXIS2_PLACEMENT_3D ( 'NONE', #44398, #84962, #54226 ) ;
#25096=DIRECTION ( 'NONE',  ( 0.000000000000000000, 1.000000000000000000, 0.000000000000000000 ) ) ;
#25097=EDGE_LOOP ( 'NONE', ( #72914, #68379 ) ) ;
#25098=ORIENTED_EDGE ( 'NONE', *, *, #110774, .F. ) ;
#25099=DIRECTION ( 'NONE',  ( -0.000000000000000000, 1.000000000000000000, -0.000000000000000000 ) ) ;
#25100=PLANE ( 'NONE',  #89770 ) ;
#25101=ORIENTED_EDGE ( 'NONE', *, *, #13443, .F. ) ;
#25102=VECTOR ( 'NONE', #53131, 1000.000000000000000 ) ;
#25103=CARTESIAN_POINT ( 'NONE',  ( 9.999999999999912959, 2.500000000000000000, -5.022947341949754119 ) ) ;
#25104=CARTESIAN_POINT ( 'NONE',  ( 11.89999999999990798, 2.500000000000000000, 4.576537180435972019 ) ) ;
#25105=ORIENTED_EDGE ( 'NONE', *, *, #62877, .F. ) ;
#25106=CIRCLE ( 'NONE', #60643, 0.06509327318403745899 ) ;
#25107=CARTESIAN_POINT ( 'NONE',  ( 12.69999999999990159, 12.50000000000000000, 4.611443907251934426 ) ) ;
#25108=LINE ( 'NONE', #25754, #89015 ) ;
#25109=AXIS2_PLACEMENT_3D ( 'NONE', #18326, #48438, #88342 ) ;
#25110=EDGE_CURVE ( 'NONE', #21005, #99549, #30023, .T. ) ;
#25111=DIRECTION ( 'NONE',  ( 0.000000000000000000, 0.000000000000000000, 1.000000000000000000 ) ) ;
#25112=CARTESIAN_POINT ( 'NONE',  ( -9.999999999999971578, 2.500000000000000000, -4.230127018922197557 ) ) ;
#25113=DIRECTION ( 'NONE',  ( 0.000000000000000000, 0.000000000000000000, 1.000000000000000000 ) ) ;
#25114=CARTESIAN_POINT ( 'NONE',  ( 7.049999999999926992, 2.500000000000000000, 2.165063509461097713 ) ) ;
#25115=VECTOR ( 'NONE', #12995, 1000.000000000000000 ) ;
#25116=ORIENTED_EDGE ( 'NONE', *, *, #43207, .F. ) ;
#25117=EDGE_LOOP ( 'NONE', ( #103880, #14609 ) ) ;
#25118=ORIENTED_EDGE ( 'NONE', *, *, #112050, .F. ) ;
#25119=ORIENTED_EDGE ( 'NONE', *, *, #126365, .F. ) ;
#25120=AXIS2_PLACEMENT_3D ( 'NONE', #62796, #32706, #71305 ) ;
#25121=CARTESIAN_POINT ( 'NONE',  ( -10.00000000000000533, 2.500000000000000000, 5.022947341949748790 ) ) ;
#25122=FACE_OUTER_BOUND ( 'NONE', #52620, .T. ) ;
#25123=CARTESIAN_POINT ( 'NONE',  ( 14.19999999999989626, 2.500000000000000000, -0.1000000000000022815 ) ) ;
#25124=VERTEX_POINT ( 'NONE', #106878 ) ;
#25125=ADVANCED_FACE ( 'NONE', ( #66949 ), #71880, .T. ) ;
#25126=FACE_BOUND ( 'NONE', #81172, .T. ) ;
#25127=FACE_OUTER_BOUND ( 'NONE', #66959, .T. ) ;
#25128=PLANE ( 'NONE',  #6180 ) ;
#25129=FACE_OUTER_BOUND ( 'NONE', #55897, .T. ) ;
#25131=DIRECTION ( 'NONE',  ( -4.274815082592931898E-19, -0.9999939076577903929, -0.003490651415223739937 ) ) ;
#25132=CARTESIAN_POINT ( 'NONE',  ( 11.44999999999990514, 2.500000000000000000, -6.148780366869526226 ) ) ;
#25133=DIRECTION ( 'NONE',  ( 0.000000000000000000, 1.000000000000000000, 0.000000000000000000 ) ) ;
#25134=CARTESIAN_POINT ( 'NONE',  ( -2.100000000000033396, 12.50000000000000000, 0.6928203230275494784 ) ) ;
#25135=CARTESIAN_POINT ( 'NONE',  ( -2.300000000000032685, 2.500000000000000000, -4.676537180435978769 ) ) ;
#25136=DIRECTION ( 'NONE',  ( 0.000000000000000000, 1.000000000000000000, 0.000000000000000000 ) ) ;
#25137=ORIENTED_EDGE ( 'NONE', *, *, #103485, .F. ) ;
#25138=EDGE_LOOP ( 'NONE', ( #48491, #46512 ) ) ;
#25139=ORIENTED_EDGE ( 'NONE', *, *, #119586, .F. ) ;
#25140=ORIENTED_EDGE ( 'NONE', *, *, #102342, .F. ) ;
#25141=CARTESIAN_POINT ( 'NONE',  ( 12.09999999999990550, 12.50000000000000000, 4.957854068765711553 ) ) ;
#25142=EDGE_LOOP ( 'NONE', ( #11665, #5207 ) ) ;
#25143=AXIS2_PLACEMENT_3D ( 'NONE', #95372, #116280, #5677 ) ;
#25144=CARTESIAN_POINT ( 'NONE',  ( -14.14999999999998792, 2.500000000000000000, 2.857883832488652853 ) ) ;
#25145=EDGE_LOOP ( 'NONE', ( #67105, #15185 ) ) ;
#25146=ORIENTED_EDGE ( 'NONE', *, *, #91573, .F. ) ;
#25147=EDGE_CURVE ( 'NONE', #45548, #34729, #111571, .T. ) ;
#25148=AXIS2_PLACEMENT_3D ( 'NONE', #43444, #23790, #64348 ) ;
#25149=AXIS2_PLACEMENT_3D ( 'NONE', #93853, #4160, #112854 ) ;
#25150=CARTESIAN_POINT ( 'NONE',  ( 10.89704209839471716, -1.500000000000189626, 8.980393934824014934 ) ) ;
#25151=DIRECTION ( 'NONE',  ( 0.000000000000000000, 1.000000000000000000, 0.000000000000000000 ) ) ;
#25152=FACE_OUTER_BOUND ( 'NONE', #126018, .T. ) ;
#25153=DIRECTION ( 'NONE',  ( 0.000000000000000000, 0.000000000000000000, 1.000000000000000000 ) ) ;
#25154=ORIENTED_EDGE ( 'NONE', *, *, #98015, .T. ) ;
#25155=EDGE_CURVE ( 'NONE', #95676, #54254, #17465, .T. ) ;
#25156=VERTEX_POINT ( 'NONE', #25107 ) ;
#25157=ORIENTED_EDGE ( 'NONE', *, *, #63597, .T. ) ;
#25158=CARTESIAN_POINT ( 'NONE',  ( 3.749999999999942268, 2.500000000000000000, -1.472243186433550122 ) ) ;
#25159=ORIENTED_EDGE ( 'NONE', *, *, #25968, .F. ) ;
#25160=EDGE_CURVE ( 'NONE', #7810, #106597, #96896, .T. ) ;
#25161=DIRECTION ( 'NONE',  ( 0.000000000000000000, 0.000000000000000000, -1.000000000000000000 ) ) ;
#25162=EDGE_CURVE ( 'NONE', #96782, #117692, #104941, .T. ) ;
#25163=ADVANCED_FACE ( 'NONE', ( #15263 ), #4943, .T. ) ;
#25165=EDGE_CURVE ( 'NONE', #25630, #60755, #124088, .T. ) ;
#25166=ORIENTED_EDGE ( 'NONE', *, *, #95816, .F. ) ;
#25167=CARTESIAN_POINT ( 'NONE',  ( 5.849999999999933031, 2.500000000000000000, 7.188010851410848723 ) ) ;
#25168=CARTESIAN_POINT ( 'NONE',  ( 2.899999999999946620, 2.500000000000000000, -0.7928203230275543412 ) ) ;
#25169=DIRECTION ( 'NONE',  ( 0.000000000000000000, -0.000000000000000000, 1.000000000000000000 ) ) ;
#25170=CARTESIAN_POINT ( 'NONE',  ( -1.650000000000034772, 2.500000000000000000, 1.472243186433545459 ) ) ;
#25171=CARTESIAN_POINT ( 'NONE',  ( -4.600000000000028955, 2.500000000000000000, -4.330127018922201643 ) ) ;
#25172=ADVANCED_FACE ( 'NONE', ( #86600 ), #86428, .T. ) ;
#25174=CARTESIAN_POINT ( 'NONE',  ( -6.250000000000015987, 12.50000000000000000, 1.472243186433545459 ) ) ;
#25175=ADVANCED_FACE ( 'NONE', ( #55854 ), #78138, .T. ) ;
#25176=CIRCLE ( 'NONE', #98329, 0.09999999999999999167 ) ;
#25177=ADVANCED_FACE ( 'NONE', ( #95787 ), #75487, .T. ) ;
#25178=VERTEX_POINT ( 'NONE', #4807 ) ;
#25179=CARTESIAN_POINT ( 'NONE',  ( -1.250000000000037970, 12.50000000000000000, 2.857883832488649301 ) ) ;
#25180=ORIENTED_EDGE ( 'NONE', *, *, #70008, .F. ) ;
#25181=CARTESIAN_POINT ( 'NONE',  ( 4.999999999999935163, 2.500000000000000000, 3.737306695894644371 ) ) ;
#25182=DIRECTION ( 'NONE',  ( 0.000000000000000000, -0.000000000000000000, 1.000000000000000000 ) ) ;
#25183=CARTESIAN_POINT ( 'NONE',  ( 4.599999999999936584, 2.500000000000000000, 4.330127018922196314 ) ) ;
#25184=CARTESIAN_POINT ( 'NONE',  ( -6.450000000000019718, 2.500000000000000000, -1.918653347947326004 ) ) ;
#25185=ORIENTED_EDGE ( 'NONE', *, *, #114820, .F. ) ;
#25186=AXIS2_PLACEMENT_3D ( 'NONE', #100574, #101233, #80315 ) ;
#25188=CARTESIAN_POINT ( 'NONE',  ( 7.899999999999923084, 2.500000000000000000, -0.6928203230275542523 ) ) ;
#25189=ORIENTED_EDGE ( 'NONE', *, *, #119423, .T. ) ;
#25190=ORIENTED_EDGE ( 'NONE', *, *, #35160, .T. ) ;
#25191=ORIENTED_EDGE ( 'NONE', *, *, #64480, .F. ) ;
#25192=CARTESIAN_POINT ( 'NONE',  ( -0.6000000000000388356, 12.50000000000000000, 3.983716857408420964 ) ) ;
#25193=DIRECTION ( 'NONE',  ( 0.000000000000000000, 0.000000000000000000, 1.000000000000000000 ) ) ;
#25195=FACE_OUTER_BOUND ( 'NONE', #50764, .T. ) ;
#25197=AXIS2_PLACEMENT_3D ( 'NONE', #59414, #128800, #88171 ) ;
#25198=CARTESIAN_POINT ( 'NONE',  ( -10.84999999999999964, 2.500000000000000000, 7.088010851410848190 ) ) ;
#25199=CARTESIAN_POINT ( 'NONE',  ( 7.899999999999923084, 2.500000000000000000, 0.6928203230275494784 ) ) ;
#25200=VECTOR ( 'NONE', #96720, 1000.000000000000000 ) ;
#25201=EDGE_LOOP ( 'NONE', ( #61771, #93695 ) ) ;
#25202=CARTESIAN_POINT ( 'NONE',  ( 5.849999999999935696, 12.50000000000000000, -7.253104124594891289 ) ) ;
#25203=ORIENTED_EDGE ( 'NONE', *, *, #73606, .F. ) ;
#25204=CARTESIAN_POINT ( 'NONE',  ( 5.599999999999934808, 12.50000000000000000, -3.918623584224389056 ) ) ;
#25205=CARTESIAN_POINT ( 'NONE',  ( 8.749999999999923617, 2.500000000000000000, -7.188010851410854052 ) ) ;
#25206=ADVANCED_FACE ( 'NONE', ( #14623 ), #76151, .T. ) ;
#25207=DIRECTION ( 'NONE',  ( -0.000000000000000000, 1.000000000000000000, -0.000000000000000000 ) ) ;
#25208=ORIENTED_EDGE ( 'NONE', *, *, #12449, .T. ) ;
#25209=EDGE_CURVE ( 'NONE', #53781, #97017, #105616, .T. ) ;
#25210=EDGE_CURVE ( 'NONE', #57482, #110807, #109526, .T. ) ;
#25211=CARTESIAN_POINT ( 'NONE',  ( -4.150000000000025224, 2.500000000000000000, 7.188010851410848723 ) ) ;
#25212=FACE_OUTER_BOUND ( 'NONE', #68246, .T. ) ;
#25213=ORIENTED_EDGE ( 'NONE', *, *, #15384, .F. ) ;
#25214=ADVANCED_FACE ( 'NONE', ( #6726 ), #25894, .T. ) ;
#25216=ORIENTED_EDGE ( 'NONE', *, *, #64344, .F. ) ;
#25218=PLANE ( 'NONE',  #117704 ) ;
#25219=VECTOR ( 'NONE', #14690, 1000.000000000000000 ) ;
#25220=CONICAL_SURFACE ( 'NONE', #29451, 0.1000000000000002554, 0.003490658503988666988 ) ;
#25221=AXIS2_PLACEMENT_3D ( 'NONE', #121437, #11495, #13415 ) ;
#25222=ORIENTED_EDGE ( 'NONE', *, *, #91988, .F. ) ;
#25223=DIRECTION ( 'NONE',  ( 0.000000000000000000, 1.000000000000000000, 0.000000000000000000 ) ) ;
#25224=DIRECTION ( 'NONE',  ( -0.000000000000000000, 1.000000000000000000, -0.000000000000000000 ) ) ;
#25225=CARTESIAN_POINT ( 'NONE',  ( -11.84999999999999787, 12.50000000000000000, -1.818653347947321919 ) ) ;
#25226=ORIENTED_EDGE ( 'NONE', *, *, #25418, .T. ) ;
#25227=CIRCLE ( 'NONE', #33659, 0.06509327318403745899 ) ;
#25228=FACE_BOUND ( 'NONE', #44140, .T. ) ;
#25229=CARTESIAN_POINT ( 'NONE',  ( -9.200000000000009948, 12.50000000000000000, -4.330127018922197202 ) ) ;
#25230=ORIENTED_EDGE ( 'NONE', *, *, #62198, .T. ) ;
#25231=VECTOR ( 'NONE', #10806, 1000.000000000000000 ) ;
#25232=DIRECTION ( 'NONE',  ( -0.000000000000000000, 1.000000000000000000, -0.000000000000000000 ) ) ;
#25233=DIRECTION ( 'NONE',  ( -4.274815082592931898E-19, -0.9999939076577903929, -0.003490651415223739937 ) ) ;
#25234=EDGE_CURVE ( 'NONE', #121575, #80079, #47342, .T. ) ;
#25235=ORIENTED_EDGE ( 'NONE', *, *, #13021, .F. ) ;
#25236=ORIENTED_EDGE ( 'NONE', *, *, #38957, .F. ) ;
#25237=ORIENTED_EDGE ( 'NONE', *, *, #110256, .F. ) ;
#25238=DIRECTION ( 'NONE',  ( 0.000000000000000000, -0.9999939076577903929, 0.003490651415223739937 ) ) ;
#25239=CARTESIAN_POINT ( 'NONE',  ( 14.14999999999989555, 12.50000000000000000, 2.099970236277060032 ) ) ;
#25240=FACE_OUTER_BOUND ( 'NONE', #20377, .T. ) ;
#25241=FACE_BOUND ( 'NONE', #75179, .T. ) ;
#25242=ORIENTED_EDGE ( 'NONE', *, *, #63262, .T. ) ;
#25244=CARTESIAN_POINT ( 'NONE',  ( -9.800000000000004263, 2.500000000000000000, -0.4464101615137783252 ) ) ;
#25245=FACE_OUTER_BOUND ( 'NONE', #128541, .T. ) ;
#25246=CARTESIAN_POINT ( 'NONE',  ( -5.400000000000020783, 2.500000000000000000, 5.022947341949748790 ) ) ;
#25247=EDGE_CURVE ( 'NONE', #63253, #47460, #88591, .T. ) ;
#25248=CARTESIAN_POINT ( 'NONE',  ( 5.399999999999932854, 12.50000000000000000, 4.957854068765711553 ) ) ;
#25249=CARTESIAN_POINT ( 'NONE',  ( -2.100000000000034284, 12.50000000000000000, -4.395220292106239768 ) ) ;
#25250=CARTESIAN_POINT ( 'NONE',  ( -8.550000000000009592, 2.500000000000000000, 6.841600689897072485 ) ) ;
#25251=DIRECTION ( 'NONE',  ( 0.000000000000000000, 1.000000000000000000, 0.000000000000000000 ) ) ;
#25252=CONICAL_SURFACE ( 'NONE', #23128, 0.1000000000000002554, 0.003490658503988666988 ) ;
#25253=CONICAL_SURFACE ( 'NONE', #108884, 0.1000000000000000472, 0.003490658503988666988 ) ;
#25254=DIRECTION ( 'NONE',  ( -0.000000000000000000, 1.000000000000000000, -0.000000000000000000 ) ) ;
#25255=EDGE_LOOP ( 'NONE', ( #104408, #724 ) ) ;
#25256=ORIENTED_EDGE ( 'NONE', *, *, #40464, .F. ) ;
#25257=ORIENTED_EDGE ( 'NONE', *, *, #94940, .F. ) ;
#25258=EDGE_LOOP ( 'NONE', ( #21103, #50309, #21432, #76213 ) ) ;
#25259=ORIENTED_EDGE ( 'NONE', *, *, #3748, .T. ) ;
#25260=CARTESIAN_POINT ( 'NONE',  ( -0.8500000000000382805, 2.500000000000000000, -2.857883832488653741 ) ) ;
#25261=CARTESIAN_POINT ( 'NONE',  ( 6.249999999999932498, 2.500000000000000000, -2.957883832488653830 ) ) ;
#25262=ORIENTED_EDGE ( 'NONE', *, *, #64650, .F. ) ;
#25263=EDGE_CURVE ( 'NONE', #46243, #23743, #15407, .T. ) ;
#25264=FACE_BOUND ( 'NONE', #77563, .T. ) ;
#25265=CARTESIAN_POINT ( 'NONE',  ( -1.250000000000001110, 2.500000000000000000, -2.065063509461102065 ) ) ;
#25266=CIRCLE ( 'NONE', #67108, 0.09999999999999982514 ) ;
#25267=LINE ( 'NONE', #56660, #65739 ) ;
#25268=ORIENTED_EDGE ( 'NONE', *, *, #89471, .T. ) ;
#25269=CARTESIAN_POINT ( 'NONE',  ( 2.499999999999945377, 2.500000000000000000, 5.122947341949749323 ) ) ;
#25270=ADVANCED_FACE ( 'NONE', ( #40759 ), #9337, .T. ) ;
#25271=CARTESIAN_POINT ( 'NONE',  ( -14.99999999999998224, 2.500000000000000000, -0.6928203230275519209 ) ) ;
#25273=ORIENTED_EDGE ( 'NONE', *, *, #44977, .T. ) ;
#25274=DIRECTION ( 'NONE',  ( -0.000000000000000000, -1.000000000000000000, -0.000000000000000000 ) ) ;
#25275=CONICAL_SURFACE ( 'NONE', #142, 0.09999999999999982514, 0.003490658503988666988 ) ;
#25276=ORIENTED_EDGE ( 'NONE', *, *, #41922, .F. ) ;
#25277=AXIS2_PLACEMENT_3D ( 'NONE', #113641, #6236, #5593 ) ;
#25278=EDGE_LOOP ( 'NONE', ( #110644, #61717, #109858, #39983 ) ) ;
#25279=VERTEX_POINT ( 'NONE', #117994 ) ;
#25280=CARTESIAN_POINT ( 'NONE',  ( -5.600000000000023626, 2.500000000000000000, -4.676537180435977881 ) ) ;
#25281=DIRECTION ( 'NONE',  ( -0.000000000000000000, -1.000000000000000000, -0.000000000000000000 ) ) ;
#25282=DIRECTION ( 'NONE',  ( 0.000000000000000000, 0.000000000000000000, 1.000000000000000000 ) ) ;
#25283=ORIENTED_EDGE ( 'NONE', *, *, #58897, .T. ) ;
#25284=DIRECTION ( 'NONE',  ( -0.000000000000000000, -1.000000000000000000, -0.000000000000000000 ) ) ;
#25285=AXIS2_PLACEMENT_3D ( 'NONE', #27328, #57464, #58113 ) ;
#25286=PLANE ( 'NONE',  #24008 ) ;
#25287=ADVANCED_FACE ( 'NONE', ( #120582 ), #82348, .T. ) ;
#25288=CARTESIAN_POINT ( 'NONE',  ( 5.849999999999931255, 2.500000000000000000, 2.857883832488649301 ) ) ;
#25289=AXIS2_PLACEMENT_3D ( 'NONE', #13994, #53941, #112864 ) ;
#25291=CARTESIAN_POINT ( 'NONE',  ( -5.000000000000023093, 2.500000000000000000, 4.922947341949748257 ) ) ;
#25292=DIRECTION ( 'NONE',  ( -0.000000000000000000, -1.000000000000000000, -0.000000000000000000 ) ) ;
#25293=EDGE_LOOP ( 'NONE', ( #18299, #105159, #8244, #89343 ) ) ;
#25294=DIRECTION ( 'NONE',  ( 0.000000000000000000, 0.000000000000000000, 1.000000000000000000 ) ) ;
#25295=EDGE_CURVE ( 'NONE', #8330, #123664, #18511, .T. ) ;
#25296=ORIENTED_EDGE ( 'NONE', *, *, #95109, .F. ) ;
#25297=EDGE_LOOP ( 'NONE', ( #105651, #57124, #64140, #119678 ) ) ;
#25298=CARTESIAN_POINT ( 'NONE',  ( -12.89999999999999147, 12.50000000000000000, -4.265033745738161741 ) ) ;
#25300=EDGE_CURVE ( 'NONE', #87351, #118459, #108812, .T. ) ;
#25301=CARTESIAN_POINT ( 'NONE',  ( -2.500000000000030642, 2.500000000000000000, -0.6928203230275541413 ) ) ;
#25302=DIRECTION ( 'NONE',  ( 0.000000000000000000, 0.000000000000000000, 1.000000000000000000 ) ) ;
#25304=EDGE_CURVE ( 'NONE', #96622, #99498, #13268, .T. ) ;
#25305=DIRECTION ( 'NONE',  ( 0.000000000000000000, -0.000000000000000000, 1.000000000000000000 ) ) ;
#25306=ADVANCED_FACE ( 'NONE', ( #68250 ), #63459, .T. ) ;
#25307=EDGE_LOOP ( 'NONE', ( #80987, #16208 ) ) ;
#25308=ORIENTED_EDGE ( 'NONE', *, *, #67183, .T. ) ;
#25309=DIRECTION ( 'NONE',  ( 0.000000000000000000, 1.000000000000000000, 0.000000000000000000 ) ) ;
#25310=CARTESIAN_POINT ( 'NONE',  ( 9.599999999999914380, 12.50000000000000000, -5.088040615133791356 ) ) ;
#25311=EDGE_CURVE ( 'NONE', #98287, #19378, #69538, .T. ) ;
#25312=CIRCLE ( 'NONE', #117321, 0.06509327318403745899 ) ;
#25313=CARTESIAN_POINT ( 'NONE',  ( 14.59999999999989484, 2.500000000000000000, -0.5928203230275541635 ) ) ;
#25314=ORIENTED_EDGE ( 'NONE', *, *, #51656, .T. ) ;
#25315=ORIENTED_EDGE ( 'NONE', *, *, #51539, .F. ) ;
#25316=CIRCLE ( 'NONE', #125662, 0.06509327318403745899 ) ;
#25317=CONICAL_SURFACE ( 'NONE', #40019, 0.1000000000000002554, 0.003490658503988666988 ) ;
#25319=DIRECTION ( 'NONE',  ( -4.274815082592931898E-19, -0.9999939076577903929, -0.003490651415223739937 ) ) ;
#25320=EDGE_CURVE ( 'NONE', #66380, #106765, #752, .T. ) ;
#25321=VERTEX_POINT ( 'NONE', #89826 ) ;
#25322=DIRECTION ( 'NONE',  ( 0.000000000000000000, 0.000000000000000000, 1.000000000000000000 ) ) ;
#25323=EDGE_CURVE ( 'NONE', #10983, #71602, #128420, .T. ) ;
#25324=CIRCLE ( 'NONE', #104736, 0.06509327318403745899 ) ;
#25325=EDGE_CURVE ( 'NONE', #76363, #126865, #122148, .T. ) ;
#25326=CARTESIAN_POINT ( 'NONE',  ( 11.69999999999990514, 2.500000000000000000, -2.276824562219559311E-15 ) ) ;
#25328=DIRECTION ( 'NONE',  ( 0.000000000000000000, 0.000000000000000000, 1.000000000000000000 ) ) ;
#25330=CARTESIAN_POINT ( 'NONE',  ( 4.149999999999936406, 2.500000000000000000, 6.495190528383297135 ) ) ;
#25331=VECTOR ( 'NONE', #26467, 1000.000000000000000 ) ;
#25333=ADVANCED_FACE ( 'NONE', ( #143 ), #25997, .T. ) ;
#25334=EDGE_LOOP ( 'NONE', ( #40282, #121366, #123844, #71481 ) ) ;
#25335=FACE_OUTER_BOUND ( 'NONE', #115783, .T. ) ;
#25336=DIRECTION ( 'NONE',  ( 0.000000000000000000, 0.000000000000000000, -1.000000000000000000 ) ) ;
#25337=VERTEX_POINT ( 'NONE', #47989 ) ;
#25338=ORIENTED_EDGE ( 'NONE', *, *, #92069, .F. ) ;
#25339=PLANE ( 'NONE',  #27459 ) ;
#25340=CARTESIAN_POINT ( 'NONE',  ( 9.349999999999919709, 12.50000000000000000, -6.148780366869526226 ) ) ;
#25341=CARTESIAN_POINT ( 'NONE',  ( 8.149999999999920419, 2.500000000000000000, -1.718653347947325827 ) ) ;
#25342=DIRECTION ( 'NONE',  ( 0.000000000000000000, 0.000000000000000000, 1.000000000000000000 ) ) ;
#25343=CARTESIAN_POINT ( 'NONE',  ( -9.550000000000006040, 12.50000000000000000, 2.230156782645134950 ) ) ;
#25344=DIRECTION ( 'NONE',  ( 0.000000000000000000, -0.000000000000000000, 1.000000000000000000 ) ) ;
#25345=CARTESIAN_POINT ( 'NONE',  ( -7.500000000000001776, -1.500000000000000000, -9.999999999999998224 ) ) ;
#25346=DIRECTION ( 'NONE',  ( 0.000000000000000000, -0.000000000000000000, 1.000000000000000000 ) ) ;
#25347=CARTESIAN_POINT ( 'NONE',  ( -1.050000000000038236, 2.500000000000000000, -6.048780366869526581 ) ) ;
#25348=FACE_OUTER_BOUND ( 'NONE', #19120, .T. ) ;
#25350=CIRCLE ( 'NONE', #83847, 0.09999999999999982514 ) ;
#25351=ORIENTED_EDGE ( 'NONE', *, *, #106176, .F. ) ;
#25352=AXIS2_PLACEMENT_3D ( 'NONE', #87950, #48061, #222 ) ;
#25354=ORIENTED_EDGE ( 'NONE', *, *, #19270, .T. ) ;
#25355=LINE ( 'NONE', #75753, #58317 ) ;
#25356=DIRECTION ( 'NONE',  ( 0.000000000000000000, 1.000000000000000000, 0.000000000000000000 ) ) ;
#25357=DIRECTION ( 'NONE',  ( 0.000000000000000000, 0.000000000000000000, 1.000000000000000000 ) ) ;
#25359=AXIS2_PLACEMENT_3D ( 'NONE', #5856, #16313, #75898 ) ;
#25360=EDGE_LOOP ( 'NONE', ( #55464, #55955 ) ) ;
#25361=CARTESIAN_POINT ( 'NONE',  ( -11.89999999999999503, 12.50000000000000000, 3.983716857408420076 ) ) ;
#25362=ADVANCED_FACE ( 'NONE', ( #87878 ), #30291, .T. ) ;
#25363=EDGE_CURVE ( 'NONE', #97929, #81732, #99154, .T. ) ;
#25364=CARTESIAN_POINT ( 'NONE',  ( 1.049999999999952083, 2.500000000000000000, 6.841600689897072485 ) ) ;
#25365=LINE ( 'NONE', #44373, #41309 ) ;
#25366=EDGE_LOOP ( 'NONE', ( #93144, #38923 ) ) ;
#25367=DIRECTION ( 'NONE',  ( 0.000000000000000000, 0.000000000000000000, 1.000000000000000000 ) ) ;
#25368=AXIS2_PLACEMENT_3D ( 'NONE', #101228, #11547, #42983 ) ;
#25369=ORIENTED_EDGE ( 'NONE', *, *, #94511, .T. ) ;
#25370=ADVANCED_FACE ( 'NONE', ( #127818 ), #9265, .T. ) ;
#25371=AXIS2_PLACEMENT_3D ( 'NONE', #47480, #89339, #6874 ) ;
#25372=VERTEX_POINT ( 'NONE', #83248 ) ;
#25373=ORIENTED_EDGE ( 'NONE', *, *, #114585, .T. ) ;
#25374=VECTOR ( 'NONE', #61296, 1000.000000000000000 ) ;
#25375=VERTEX_POINT ( 'NONE', #52475 ) ;
#25376=DIRECTION ( 'NONE',  ( 0.000000000000000000, -0.000000000000000000, 1.000000000000000000 ) ) ;
#25377=AXIS2_PLACEMENT_3D ( 'NONE', #55370, #46187, #86089 ) ;
#25378=CARTESIAN_POINT ( 'NONE',  ( -13.09999999999999254, 12.50000000000000000, 0.3464101615137777923 ) ) ;
#25379=DIRECTION ( 'NONE',  ( -0.000000000000000000, 1.000000000000000000, -0.000000000000000000 ) ) ;
#25380=FACE_OUTER_BOUND ( 'NONE', #20379, .T. ) ;
#25382=AXIS2_PLACEMENT_3D ( 'NONE', #72782, #43332, #113337 ) ;
#25383=AXIS2_PLACEMENT_3D ( 'NONE', #105836, #16142, #98570 ) ;
#25384=LINE ( 'NONE', #3827, #10514 ) ;
#25385=VERTEX_POINT ( 'NONE', #42025 ) ;
#25386=CARTESIAN_POINT ( 'NONE',  ( 21.23528140090950345, -2.699413673072311504, -2.293764360948880476 ) ) ;
#25387=DIRECTION ( 'NONE',  ( 0.000000000000000000, 0.000000000000000000, 1.000000000000000000 ) ) ;
#25388=CARTESIAN_POINT ( 'NONE',  ( -17.50000000000000000, -1.500000000000000000, 9.000000000000001776 ) ) ;
#25389=CARTESIAN_POINT ( 'NONE',  ( 16.58100817950494843, -2.557139044001658146, 6.067820687733448182 ) ) ;
#25390=ORIENTED_EDGE ( 'NONE', *, *, #1695, .F. ) ;
#25391=ORIENTED_EDGE ( 'NONE', *, *, #111641, .T. ) ;
#25392=ORIENTED_EDGE ( 'NONE', *, *, #9273, .T. ) ;
#25393=DIRECTION ( 'NONE',  ( 0.000000000000000000, 0.000000000000000000, 1.000000000000000000 ) ) ;
#25394=FACE_OUTER_BOUND ( 'NONE', #46699, .T. ) ;
#25395=DIRECTION ( 'NONE',  ( 0.000000000000000000, -0.9999939076577903929, 0.003490651415223739937 ) ) ;
#25396=FACE_BOUND ( 'NONE', #128836, .T. ) ;
#25397=CARTESIAN_POINT ( 'NONE',  ( -11.89999999999999680, 12.50000000000000000, 0.2813168883297402778 ) ) ;
#25398=DIRECTION ( 'NONE',  ( 0.000000000000000000, 0.000000000000000000, 1.000000000000000000 ) ) ;
#25399=DIRECTION ( 'NONE',  ( 0.000000000000000000, 1.000000000000000000, 0.000000000000000000 ) ) ;
#25400=LINE ( 'NONE', #23485, #95988 ) ;
#25401=EDGE_CURVE ( 'NONE', #97177, #67035, #30120, .T. ) ;
#25402=CIRCLE ( 'NONE', #50541, 0.1000000000000002554 ) ;
#25403=AXIS2_PLACEMENT_3D ( 'NONE', #90069, #49533, #69143 ) ;
#25404=DIRECTION ( 'NONE',  ( 0.000000000000000000, -0.000000000000000000, 1.000000000000000000 ) ) ;
#25405=CIRCLE ( 'NONE', #115278, 0.06509327318403743123 ) ;
#25407=CARTESIAN_POINT ( 'NONE',  ( -1.450000000000035927, 12.50000000000000000, -1.883746621131363597 ) ) ;
#25408=CIRCLE ( 'NONE', #42160, 0.06509327318403745899 ) ;
#25409=DIRECTION ( 'NONE',  ( 0.000000000000000000, 0.000000000000000000, 1.000000000000000000 ) ) ;
#25410=AXIS2_PLACEMENT_3D ( 'NONE', #19349, #96614, #116903 ) ;
#25411=ORIENTED_EDGE ( 'NONE', *, *, #48625, .T. ) ;
#25412=VERTEX_POINT ( 'NONE', #21745 ) ;
#25413=ORIENTED_EDGE ( 'NONE', *, *, #106634, .F. ) ;
#25414=EDGE_LOOP ( 'NONE', ( #26027, #125427 ) ) ;
#25415=CONICAL_SURFACE ( 'NONE', #73538, 0.1000000000000000472, 0.003490658503988666988 ) ;
#25416=EDGE_CURVE ( 'NONE', #15697, #77313, #30930, .T. ) ;
#25417=CARTESIAN_POINT ( 'NONE',  ( 9.599999999999914380, 12.50000000000000000, 3.702399969078682407 ) ) ;
#25418=EDGE_CURVE ( 'NONE', #34661, #53613, #38531, .T. ) ;
#25419=FACE_BOUND ( 'NONE', #117441, .T. ) ;
#25420=CARTESIAN_POINT ( 'NONE',  ( -6.900000000000015454, 12.50000000000000000, 3.983716857408420076 ) ) ;
#25422=EDGE_LOOP ( 'NONE', ( #88033, #75677, #101451, #94348 ) ) ;
#25423=CARTESIAN_POINT ( 'NONE',  ( 76.45227062019213804, 3.905198618281777723, 5.870121734766100552 ) ) ;
#25424=EDGE_CURVE ( 'NONE', #1183, #106661, #121867, .T. ) ;
#25425=CARTESIAN_POINT ( 'NONE',  ( -1.650000000000035660, 12.50000000000000000, 2.857883832488649301 ) ) ;
#25426=VERTEX_POINT ( 'NONE', #112057 ) ;
#25427=DIRECTION ( 'NONE',  ( 0.000000000000000000, 0.000000000000000000, 1.000000000000000000 ) ) ;
#25428=CARTESIAN_POINT ( 'NONE',  ( 7.049999999999930544, 2.500000000000000000, -6.495190528383302464 ) ) ;
#25429=ADVANCED_FACE ( 'NONE', ( #22401 ), #63556, .T. ) ;
#25430=VERTEX_POINT ( 'NONE', #21085 ) ;
#25431=DIRECTION ( 'NONE',  ( 0.000000000000000000, -0.000000000000000000, 1.000000000000000000 ) ) ;
#25432=DIRECTION ( 'NONE',  ( 0.000000000000000000, 0.000000000000000000, -1.000000000000000000 ) ) ;
#25433=AXIS2_PLACEMENT_3D ( 'NONE', #62740, #33288, #45674 ) ;
#25434=AXIS2_PLACEMENT_3D ( 'NONE', #64311, #26335, #126468 ) ;
#25435=VERTEX_POINT ( 'NONE', #61677 ) ;
#25436=LINE ( 'NONE', #104027, #17543 ) ;
#25437=DIRECTION ( 'NONE',  ( 0.000000000000000000, 0.000000000000000000, -1.000000000000000000 ) ) ;
#25438=DIRECTION ( 'NONE',  ( -0.000000000000000000, 1.000000000000000000, -0.000000000000000000 ) ) ;
#25439=EDGE_LOOP ( 'NONE', ( #124406, #19710, #15767, #109192 ) ) ;
#25440=VERTEX_POINT ( 'NONE', #62319 ) ;
#25442=AXIS2_PLACEMENT_3D ( 'NONE', #67224, #57450, #7682 ) ;
#25443=ORIENTED_EDGE ( 'NONE', *, *, #125046, .F. ) ;
#25444=CARTESIAN_POINT ( 'NONE',  ( 4.349999999999940137, 2.500000000000000000, -2.411473670974877859 ) ) ;
#25445=AXIS2_PLACEMENT_3D ( 'NONE', #103091, #95212, #4872 ) ;
#25446=CARTESIAN_POINT ( 'NONE',  ( -12.29999999999999538, 12.50000000000000000, -4.676537180435976104 ) ) ;
#25447=CONICAL_SURFACE ( 'NONE', #57044, 0.09999999999999982514, 0.003490658503988666988 ) ;
#25448=EDGE_CURVE ( 'NONE', #108113, #10762, #96997, .T. ) ;
#25449=VERTEX_POINT ( 'NONE', #11262 ) ;
#25450=AXIS2_PLACEMENT_3D ( 'NONE', #80514, #120426, #77055 ) ;
#25451=CONICAL_SURFACE ( 'NONE', #42211, 0.09999999999999999167, 0.003490658503988666988 ) ;
#25453=CARTESIAN_POINT ( 'NONE',  ( -10.00000000000000355, 2.500000000000000000, -0.6928203230275541413 ) ) ;
#25454=CARTESIAN_POINT ( 'NONE',  ( -6.050000000000017586, 2.500000000000000000, 1.918653347947321564 ) ) ;
#25455=CARTESIAN_POINT ( 'NONE',  ( -1.050000000000037348, 2.500000000000000000, -2.511473670974877948 ) ) ;
#25456=EDGE_CURVE ( 'NONE', #55712, #29239, #13361, .T. ) ;
#25457=CARTESIAN_POINT ( 'NONE',  ( -7.700000000000014388, 2.500000000000000000, -0.3464101615137782364 ) ) ;
#25459=VERTEX_POINT ( 'NONE', #75988 ) ;
#25461=AXIS2_PLACEMENT_3D ( 'NONE', #5450, #63746, #125243 ) ;
#25462=ORIENTED_EDGE ( 'NONE', *, *, #101348, .T. ) ;
#25463=CARTESIAN_POINT ( 'NONE',  ( 12.94999999999990337, 12.50000000000000000, 2.165063509461097713 ) ) ;
#25464=DIRECTION ( 'NONE',  ( 0.000000000000000000, 1.000000000000000000, 0.000000000000000000 ) ) ;
#25465=VECTOR ( 'NONE', #47987, 1000.000000000000000 ) ;
#25467=VECTOR ( 'NONE', #73741, 1000.000000000000000 ) ;
#25468=EDGE_CURVE ( 'NONE', #127685, #39745, #34321, .T. ) ;
#25469=CARTESIAN_POINT ( 'NONE',  ( -9.150000000000009237, 2.500000000000000000, -2.165063509461101710 ) ) ;
#25470=EDGE_LOOP ( 'NONE', ( #105447, #57512, #79101, #80008 ) ) ;
#25471=VERTEX_POINT ( 'NONE', #17026 ) ;
#25472=EDGE_CURVE ( 'NONE', #14841, #50907, #86611, .T. ) ;
#25473=ORIENTED_EDGE ( 'NONE', *, *, #20758, .F. ) ;
#25474=EDGE_CURVE ( 'NONE', #37222, #107667, #42747, .T. ) ;
#25475=DIRECTION ( 'NONE',  ( 0.000000000000000000, 0.000000000000000000, -1.000000000000000000 ) ) ;
#25476=AXIS2_PLACEMENT_3D ( 'NONE', #2225, #3533, #63748 ) ;
#25477=CARTESIAN_POINT ( 'NONE',  ( 1.249999999999952038, 12.50000000000000000, 2.922977105672686982 ) ) ;
#25478=LINE ( 'NONE', #55599, #16340 ) ;
#25479=EDGE_CURVE ( 'NONE', #83685, #96204, #19739, .T. ) ;
#25482=CARTESIAN_POINT ( 'NONE',  ( -7.500000000000015099, 2.500000000000000000, -0.6928203230275541413 ) ) ;
#25483=DIRECTION ( 'NONE',  ( 0.000000000000000000, 0.000000000000000000, 1.000000000000000000 ) ) ;
#25484=DIRECTION ( 'NONE',  ( -0.000000000000000000, -1.000000000000000000, -0.000000000000000000 ) ) ;
#25485=DIRECTION ( 'NONE',  ( -0.000000000000000000, 1.000000000000000000, -0.000000000000000000 ) ) ;
#25486=CARTESIAN_POINT ( 'NONE',  ( 11.04999999999991012, 12.50000000000000000, -1.818653347947326138 ) ) ;
#25487=EDGE_CURVE ( 'NONE', #127183, #16787, #94950, .T. ) ;
#25488=EDGE_LOOP ( 'NONE', ( #129121, #97800 ) ) ;
#25489=CARTESIAN_POINT ( 'NONE',  ( 11.04999999999991189, 2.500000000000000000, -2.511473670974877948 ) ) ;
#25490=EDGE_LOOP ( 'NONE', ( #9611, #68494 ) ) ;
#25491=ORIENTED_EDGE ( 'NONE', *, *, #47179, .T. ) ;
#25492=DIRECTION ( 'NONE',  ( -0.000000000000000000, -1.000000000000000000, -0.000000000000000000 ) ) ;
#25493=DIRECTION ( 'NONE',  ( 0.000000000000000000, 1.000000000000000000, 0.000000000000000000 ) ) ;
#25495=DIRECTION ( 'NONE',  ( 0.000000000000000000, 0.000000000000000000, 1.000000000000000000 ) ) ;
#25496=DIRECTION ( 'NONE',  ( -0.000000000000000000, -1.000000000000000000, -0.000000000000000000 ) ) ;
#25497=DIRECTION ( 'NONE',  ( -0.000000000000000000, 1.000000000000000000, -0.000000000000000000 ) ) ;
#25498=VECTOR ( 'NONE', #10299, 1000.000000000000000 ) ;
#25499=CARTESIAN_POINT ( 'NONE',  ( 2.299999999999947864, 2.500000000000000000, 3.983716857408420964 ) ) ;
#25500=VERTEX_POINT ( 'NONE', #5303 ) ;
#25501=DIRECTION ( 'NONE',  ( -0.000000000000000000, 1.000000000000000000, -0.000000000000000000 ) ) ;
#25502=CONICAL_SURFACE ( 'NONE', #35988, 0.1000000000000002554, 0.003490658503988666988 ) ;
#25503=CIRCLE ( 'NONE', #127924, 0.06509327318403745899 ) ;
#25505=ORIENTED_EDGE ( 'NONE', *, *, #57969, .T. ) ;
#25506=CIRCLE ( 'NONE', #98664, 0.06509327318403741736 ) ;
#25507=EDGE_LOOP ( 'NONE', ( #25881, #91974 ) ) ;
#25509=VERTEX_POINT ( 'NONE', #106729 ) ;
#25510=CONICAL_SURFACE ( 'NONE', #15123, 0.1000000000000002554, 0.003490658503988666988 ) ;
#25511=AXIS2_PLACEMENT_3D ( 'NONE', #106840, #25078, #37491 ) ;
#25512=VERTEX_POINT ( 'NONE', #124450 ) ;
#25513=CARTESIAN_POINT ( 'NONE',  ( 12.29999999999990123, 12.50000000000000000, 0.3464101615137735735 ) ) ;
#25514=DIRECTION ( 'NONE',  ( 0.000000000000000000, 0.000000000000000000, 1.000000000000000000 ) ) ;
#25515=AXIS2_PLACEMENT_3D ( 'NONE', #85567, #56723, #106500 ) ;
#25516=DIRECTION ( 'NONE',  ( -4.274815082592931898E-19, -0.9999939076577903929, -0.003490651415223739937 ) ) ;
#25517=EDGE_CURVE ( 'NONE', #120135, #120902, #45249, .T. ) ;
#25518=DIRECTION ( 'NONE',  ( -0.000000000000000000, 1.000000000000000000, -0.000000000000000000 ) ) ;
#25519=CARTESIAN_POINT ( 'NONE',  ( -11.69999999999999574, 12.50000000000000000, 4.330127018922196314 ) ) ;
#25520=ORIENTED_EDGE ( 'NONE', *, *, #114608, .T. ) ;
#25521=CARTESIAN_POINT ( 'NONE',  ( -1.050000000000037348, 2.500000000000000000, -2.511473670974877948 ) ) ;
#25522=CARTESIAN_POINT ( 'NONE',  ( -4.600000000000024514, 12.50000000000000000, -0.6277270498435167934 ) ) ;
#25523=DIRECTION ( 'NONE',  ( 0.000000000000000000, 0.000000000000000000, -1.000000000000000000 ) ) ;
#25524=EDGE_CURVE ( 'NONE', #71846, #21325, #101207, .T. ) ;
#25525=EDGE_LOOP ( 'NONE', ( #23361, #62837 ) ) ;
#25526=B_SPLINE_CURVE_WITH_KNOTS ( 'NONE', 3,
 ( #62483, #13353, #34315, #71641 ),
 .UNSPECIFIED., .F., .F.,
 ( 4, 4 ),
 ( 0.2000000000000000944, 0.7999999999999997113 ),
 .UNSPECIFIED. ) ;
#25527=VERTEX_POINT ( 'NONE', #37374 ) ;
#25529=FACE_OUTER_BOUND ( 'NONE', #114010, .T. ) ;
#25530=DIRECTION ( 'NONE',  ( 0.000000000000000000, -0.000000000000000000, 1.000000000000000000 ) ) ;
#25531=CIRCLE ( 'NONE', #77761, 0.06509327318403745899 ) ;
#25532=FACE_OUTER_BOUND ( 'NONE', #11559, .T. ) ;
#25533=ORIENTED_EDGE ( 'NONE', *, *, #41248, .T. ) ;
#25534=DIRECTION ( 'NONE',  ( 0.000000000000000000, 1.000000000000000000, 0.000000000000000000 ) ) ;
#25535=CARTESIAN_POINT ( 'NONE',  ( 4.599999999999936584, 12.50000000000000000, 3.637306695894644726 ) ) ;
#25536=DIRECTION ( 'NONE',  ( -0.000000000000000000, -1.000000000000000000, -0.000000000000000000 ) ) ;
#25537=PLANE ( 'NONE',  #14878 ) ;
#25538=CARTESIAN_POINT ( 'NONE',  ( -10.84999999999999964, 12.50000000000000000, 7.253104124594885960 ) ) ;
#25539=VECTOR ( 'NONE', #114423, 1000.000000000000000 ) ;
#25540=AXIS2_PLACEMENT_3D ( 'NONE', #10054, #20524, #21150 ) ;
#25541=EDGE_LOOP ( 'NONE', ( #86981, #16145 ) ) ;
#25542=DIRECTION ( 'NONE',  ( 0.000000000000000000, 0.000000000000000000, 1.000000000000000000 ) ) ;
#25543=CIRCLE ( 'NONE', #2470, 0.06509327318403745899 ) ;
#25544=ORIENTED_EDGE ( 'NONE', *, *, #114338, .F. ) ;
#25545=ORIENTED_EDGE ( 'NONE', *, *, #58877, .T. ) ;
#25546=EDGE_LOOP ( 'NONE', ( #113161, #60180, #78056, #19470 ) ) ;
#25547=DIRECTION ( 'NONE',  ( -0.000000000000000000, 1.000000000000000000, -0.000000000000000000 ) ) ;
#25548=FACE_BOUND ( 'NONE', #462, .T. ) ;
#25549=CARTESIAN_POINT ( 'NONE',  ( -9.600000000000006750, 2.500000000000000000, -0.6928203230275542523 ) ) ;
#25550=DIRECTION ( 'NONE',  ( 0.000000000000000000, 0.000000000000000000, 1.000000000000000000 ) ) ;
#25551=CONICAL_SURFACE ( 'NONE', #113300, 0.1000000000000002554, 0.003490658503988666988 ) ;
#25552=CONICAL_SURFACE ( 'NONE', #94521, 0.09999999999999982514, 0.003490658503988666988 ) ;
#25553=CARTESIAN_POINT ( 'NONE',  ( -1.650000000000034328, 2.500000000000000000, -2.165063509461101710 ) ) ;
#25554=ADVANCED_FACE ( 'NONE', ( #68095 ), #119990, .T. ) ;
#25555=VECTOR ( 'NONE', #103421, 1000.000000000000000 ) ;
#25556=AXIS2_PLACEMENT_3D ( 'NONE', #93603, #112608, #94893 ) ;
#25557=AXIS2_PLACEMENT_3D ( 'NONE', #52510, #81970, #22437 ) ;
#25559=DIRECTION ( 'NONE',  ( 0.000000000000000000, 0.000000000000000000, -1.000000000000000000 ) ) ;
#25560=CARTESIAN_POINT ( 'NONE',  ( -9.350000000000004974, 2.500000000000000000, 6.048780366869521252 ) ) ;
#25561=CARTESIAN_POINT ( 'NONE',  ( -3.750000000000027534, 2.500000000000000000, -1.372243186433550033 ) ) ;
#25563=DIRECTION ( 'NONE',  ( 0.000000000000000000, 0.000000000000000000, -1.000000000000000000 ) ) ;
#25564=ORIENTED_EDGE ( 'NONE', *, *, #44274, .F. ) ;
#25565=EDGE_CURVE ( 'NONE', #2251, #27375, #99517, .T. ) ;
#25566=DIRECTION ( 'NONE',  ( -4.274815082592931898E-19, -0.9999939076577903929, -0.003490651415223739937 ) ) ;
#25567=CARTESIAN_POINT ( 'NONE',  ( -11.64999999999999858, 12.50000000000000000, -5.737276932171709198 ) ) ;
#25568=ORIENTED_EDGE ( 'NONE', *, *, #88826, .T. ) ;
#25569=EDGE_CURVE ( 'NONE', #26682, #32011, #109618, .T. ) ;
#25570=LINE ( 'NONE', #83853, #14558 ) ;
#25571=EDGE_CURVE ( 'NONE', #31935, #70505, #79855, .T. ) ;
#25572=EDGE_LOOP ( 'NONE', ( #18150, #86791 ) ) ;
#25573=FACE_BOUND ( 'NONE', #44562, .T. ) ;
#25574=PLANE ( 'NONE',  #13757 ) ;
#25575=ORIENTED_EDGE ( 'NONE', *, *, #100963, .F. ) ;
#25576=CARTESIAN_POINT ( 'NONE',  ( 13.09999999999990195, 12.50000000000000000, 3.918623584224382839 ) ) ;
#25577=FACE_OUTER_BOUND ( 'NONE', #16915, .T. ) ;
#25578=EDGE_CURVE ( 'NONE', #11600, #3400, #108670, .T. ) ;
#25579=VERTEX_POINT ( 'NONE', #98203 ) ;
#25580=ORIENTED_EDGE ( 'NONE', *, *, #81347, .T. ) ;
#25581=ADVANCED_FACE ( 'NONE', ( #109972 ), #58937, .T. ) ;
#25583=VERTEX_POINT ( 'NONE', #128340 ) ;
#25585=CARTESIAN_POINT ( 'NONE',  ( 8.299999999999922551, 12.50000000000000000, 4.330127018922196314 ) ) ;
#25586=VECTOR ( 'NONE', #108333, 1000.000000000000000 ) ;
#25587=CARTESIAN_POINT ( 'NONE',  ( -7.500000000000015099, 2.500000000000000000, -0.7928203230275542301 ) ) ;
#25588=DIRECTION ( 'NONE',  ( -0.000000000000000000, 1.000000000000000000, -0.000000000000000000 ) ) ;
#25589=CONICAL_SURFACE ( 'NONE', #121744, 0.1000000000000002554, 0.003490658503988666988 ) ;
#25590=CARTESIAN_POINT ( 'NONE',  ( 1.049999999999954969, 2.500000000000000000, -6.841600689897077814 ) ) ;
#25591=AXIS2_PLACEMENT_3D ( 'NONE', #26164, #24228, #24872 ) ;
#25592=CIRCLE ( 'NONE', #17266, 0.1000000000000002554 ) ;
#25593=ORIENTED_EDGE ( 'NONE', *, *, #23377, .F. ) ;
#25594=AXIS2_PLACEMENT_3D ( 'NONE', #32764, #115129, #27405 ) ;
#25595=EDGE_LOOP ( 'NONE', ( #105701, #79915 ) ) ;
#25596=DIRECTION ( 'NONE',  ( 0.000000000000000000, -0.000000000000000000, 1.000000000000000000 ) ) ;
#25597=CARTESIAN_POINT ( 'NONE',  ( -1.650000000000035216, 12.50000000000000000, -1.537336459617587581 ) ) ;
#25598=CARTESIAN_POINT ( 'NONE',  ( -10.84999999999999964, 12.50000000000000000, 2.857883832488649301 ) ) ;
#25599=CONICAL_SURFACE ( 'NONE', #52805, 0.1000000000000002554, 0.003490658503988666988 ) ;
#25600=DIRECTION ( 'NONE',  ( 0.000000000000000000, 1.000000000000000000, 0.000000000000000000 ) ) ;
#25602=ORIENTED_EDGE ( 'NONE', *, *, #2874, .F. ) ;
#25603=ORIENTED_EDGE ( 'NONE', *, *, #45848, .T. ) ;
#25604=FACE_BOUND ( 'NONE', #84333, .T. ) ;
#25605=ORIENTED_EDGE ( 'NONE', *, *, #45859, .F. ) ;
#25606=CARTESIAN_POINT ( 'NONE',  ( 1.249999999999950262, 2.500000000000000000, 7.188010851410848723 ) ) ;
#25607=CARTESIAN_POINT ( 'NONE',  ( 3.299999999999942979, 2.500000000000000000, 4.430127018922196847 ) ) ;
#25608=CONICAL_SURFACE ( 'NONE', #2623, 0.1000000000000002554, 0.003490658503988666988 ) ;
#25609=EDGE_LOOP ( 'NONE', ( #100697, #63484, #35620, #93159 ) ) ;
#25610=CARTESIAN_POINT ( 'NONE',  ( 3.349999999999945466, 12.50000000000000000, -7.122917578226816815 ) ) ;
#25611=CARTESIAN_POINT ( 'NONE',  ( 9.349999999999916156, 2.500000000000000000, -2.411473670974877859 ) ) ;
#25612=ADVANCED_FACE ( 'NONE', ( #9828 ), #51046, .T. ) ;
#25613=DIRECTION ( 'NONE',  ( -0.000000000000000000, 1.000000000000000000, -0.000000000000000000 ) ) ;
#25614=DIRECTION ( 'NONE',  ( 0.000000000000000000, 0.000000000000000000, -1.000000000000000000 ) ) ;
#25616=CARTESIAN_POINT ( 'NONE',  ( 10.84999999999990905, 12.50000000000000000, 2.857883832488649301 ) ) ;
#25618=CARTESIAN_POINT ( 'NONE',  ( -0.6500000000000398792, 2.500000000000000000, -2.411473670974877859 ) ) ;
#25619=EDGE_CURVE ( 'NONE', #5316, #76556, #39947, .T. ) ;
#25620=DIRECTION ( 'NONE',  ( 0.000000000000000000, 0.000000000000000000, -1.000000000000000000 ) ) ;
#25621=EDGE_CURVE ( 'NONE', #12513, #100762, #8520, .T. ) ;
#25622=AXIS2_PLACEMENT_3D ( 'NONE', #111538, #50065, #20585 ) ;
#25623=EDGE_LOOP ( 'NONE', ( #607, #23291, #52235, #56564 ) ) ;
#25624=VERTEX_POINT ( 'NONE', #38672 ) ;
#25625=PLANE ( 'NONE',  #109781 ) ;
#25626=ORIENTED_EDGE ( 'NONE', *, *, #65456, .F. ) ;
#25627=CARTESIAN_POINT ( 'NONE',  ( 0.8499999999999557909, 2.500000000000000000, -6.495190528383302464 ) ) ;
#25628=ADVANCED_FACE ( 'NONE', ( #78595 ), #67746, .T. ) ;
#25629=ORIENTED_EDGE ( 'NONE', *, *, #4711, .F. ) ;
#25630=VERTEX_POINT ( 'NONE', #87731 ) ;
#25631=EDGE_LOOP ( 'NONE', ( #72058, #125956, #33563, #75623 ) ) ;
#25632=EDGE_CURVE ( 'NONE', #40733, #34370, #37999, .T. ) ;
#25633=FACE_OUTER_BOUND ( 'NONE', #101238, .T. ) ;
#25634=ADVANCED_FACE ( 'NONE', ( #117829 ), #55237, .T. ) ;
#25635=CIRCLE ( 'NONE', #82077, 0.06509327318403745899 ) ;
#25636=AXIS2_PLACEMENT_3D ( 'NONE', #112713, #11276, #51231 ) ;
#25637=DIRECTION ( 'NONE',  ( -0.000000000000000000, -1.000000000000000000, -0.000000000000000000 ) ) ;
#25640=CARTESIAN_POINT ( 'NONE',  ( 4.999999999999936939, 2.500000000000000000, -0.6928203230275541413 ) ) ;
#25641=DIRECTION ( 'NONE',  ( -0.000000000000000000, -1.000000000000000000, -0.000000000000000000 ) ) ;
#25642=DIRECTION ( 'NONE',  ( -0.000000000000000000, -1.000000000000000000, -0.000000000000000000 ) ) ;
#25643=EDGE_LOOP ( 'NONE', ( #109873, #39207, #110527, #87151 ) ) ;
#25644=CIRCLE ( 'NONE', #98800, 0.06509327318403745899 ) ;
#25645=CONICAL_SURFACE ( 'NONE', #105056, 0.09999999999999982514, 0.003490658503988666988 ) ;
#25646=DIRECTION ( 'NONE',  ( 0.000000000000000000, -0.9999939076577903929, 0.003490651415223739937 ) ) ;
#25648=ORIENTED_EDGE ( 'NONE', *, *, #76774, .T. ) ;
#25649=AXIS2_PLACEMENT_3D ( 'NONE', #78007, #100232, #17787 ) ;
#25650=ADVANCED_FACE ( 'NONE', ( #2 ), #67838, .T. ) ;
#25651=ORIENTED_EDGE ( 'NONE', *, *, #120409, .T. ) ;
#25652=ORIENTED_EDGE ( 'NONE', *, *, #54698, .T. ) ;
#25653=VECTOR ( 'NONE', #39580, 1000.000000000000000 ) ;
#25654=ORIENTED_EDGE ( 'NONE', *, *, #32747, .F. ) ;
#25655=DIRECTION ( 'NONE',  ( -0.000000000000000000, -1.000000000000000000, -0.000000000000000000 ) ) ;
#25656=ORIENTED_EDGE ( 'NONE', *, *, #34966, .T. ) ;
#25657=ORIENTED_EDGE ( 'NONE', *, *, #58471, .F. ) ;
#25658=AXIS2_PLACEMENT_3D ( 'NONE', #7203, #37343, #25550 ) ;
#25659=CARTESIAN_POINT ( 'NONE',  ( -0.4000000000000392131, 12.50000000000000000, -5.022947341949754119 ) ) ;
#25660=AXIS2_PLACEMENT_3D ( 'NONE', #109966, #99505, #20287 ) ;
#25661=CARTESIAN_POINT ( 'NONE',  ( -4.200000000000025935, 12.50000000000000000, -2.385244779468109755E-15 ) ) ;
#25662=DIRECTION ( 'NONE',  ( 0.000000000000000000, 1.000000000000000000, 0.000000000000000000 ) ) ;
#25663=DIRECTION ( 'NONE',  ( 0.000000000000000000, -0.000000000000000000, 1.000000000000000000 ) ) ;
#25664=AXIS2_PLACEMENT_3D ( 'NONE', #52878, #103271, #51600 ) ;
#25665=DIRECTION ( 'NONE',  ( 0.000000000000000000, 0.000000000000000000, 1.000000000000000000 ) ) ;
#25666=VECTOR ( 'NONE', #31801, 1000.000000000000000 ) ;
#25667=CONICAL_SURFACE ( 'NONE', #27718, 0.09999999999999982514, 0.003490658503988666988 ) ;
#25668=CARTESIAN_POINT ( 'NONE',  ( 7.499999999999961808, 2.500000000000000000, -4.330127018922201643 ) ) ;
#25669=ORIENTED_EDGE ( 'NONE', *, *, #72932, .T. ) ;
#25670=AXIS2_PLACEMENT_3D ( 'NONE', #14311, #4479, #52970 ) ;
#25671=DIRECTION ( 'NONE',  ( 0.000000000000000000, 0.000000000000000000, 1.000000000000000000 ) ) ;
#25672=ORIENTED_EDGE ( 'NONE', *, *, #97314, .T. ) ;
#25673=CARTESIAN_POINT ( 'NONE',  ( -12.89999999999999147, 12.50000000000000000, -5.088040615133788691 ) ) ;
#25674=ORIENTED_EDGE ( 'NONE', *, *, #41010, .F. ) ;
#25675=AXIS2_PLACEMENT_3D ( 'NONE', #72481, #120922, #62017 ) ;
#25676=CARTESIAN_POINT ( 'NONE',  ( -6.900000000000019007, 2.500000000000000000, -3.983716857408426293 ) ) ;
#25677=VERTEX_POINT ( 'NONE', #10466 ) ;
#25679=LINE ( 'NONE', #65607, #72083 ) ;
#25680=PLANE ( 'NONE',  #111220 ) ;
#25681=DIRECTION ( 'NONE',  ( -0.000000000000000000, 1.000000000000000000, -0.000000000000000000 ) ) ;
#25682=FACE_OUTER_BOUND ( 'NONE', #121917, .T. ) ;
#25683=LINE ( 'NONE', #65611, #72153 ) ;
#25684=ORIENTED_EDGE ( 'NONE', *, *, #123105, .T. ) ;
#25685=CARTESIAN_POINT ( 'NONE',  ( -2.300000000000032685, 2.500000000000000000, -4.676537180435978769 ) ) ;
#25686=DIRECTION ( 'NONE',  ( -0.000000000000000000, -1.000000000000000000, -0.000000000000000000 ) ) ;
#25687=AXIS2_PLACEMENT_3D ( 'NONE', #93597, #22304, #3923 ) ;
#25688=AXIS2_PLACEMENT_3D ( 'NONE', #123712, #62888, #102790 ) ;
#25689=CARTESIAN_POINT ( 'NONE',  ( -0.4500000000000397571, 2.500000000000000000, -2.165063509461101710 ) ) ;
#25690=DIRECTION ( 'NONE',  ( 0.000000000000000000, 1.000000000000000000, 0.000000000000000000 ) ) ;
#25691=CARTESIAN_POINT ( 'NONE',  ( 6.449999999999931788, 2.500000000000000000, -2.611473670974877592 ) ) ;
#25692=EDGE_CURVE ( 'NONE', #104247, #63955, #127043, .T. ) ;
#25693=ORIENTED_EDGE ( 'NONE', *, *, #22473, .T. ) ;
#25694=AXIS2_PLACEMENT_3D ( 'NONE', #4430, #34597, #15558 ) ;
#25695=AXIS2_PLACEMENT_3D ( 'NONE', #37994, #38668, #97555 ) ;
#25696=ORIENTED_EDGE ( 'NONE', *, *, #92089, .T. ) ;
#25697=AXIS2_PLACEMENT_3D ( 'NONE', #61390, #101954, #52853 ) ;
#25698=AXIS2_PLACEMENT_3D ( 'NONE', #25850, #34400, #74949 ) ;
#25699=UNCERTAINTY_MEASURE_WITH_UNIT (LENGTH_MEASURE( 1.000000000000000082E-05 ), #30989, 'distance_accuracy_value', 'NONE');
#25700=EDGE_LOOP ( 'NONE', ( #69401, #53825 ) ) ;
#25701=FACE_OUTER_BOUND ( 'NONE', #15688, .T. ) ;
#25702=CARTESIAN_POINT ( 'NONE',  ( -3.749999999999991562, 2.500000000000000000, 6.495190528383297135 ) ) ;
#25703=AXIS2_PLACEMENT_3D ( 'NONE', #127768, #10554, #37476 ) ;
#25704=AXIS2_PLACEMENT_3D ( 'NONE', #84299, #5084, #47609 ) ;
#25705=CONICAL_SURFACE ( 'NONE', #67435, 0.1000000000000002554, 0.003490658503988666988 ) ;
#25706=CIRCLE ( 'NONE', #90552, 0.09999999999999982514 ) ;
#25708=DIRECTION ( 'NONE',  ( 0.000000000000000000, -0.9999939076577903929, 0.003490651415223739937 ) ) ;
#25709=DIRECTION ( 'NONE',  ( 0.000000000000000000, 0.000000000000000000, -1.000000000000000000 ) ) ;
#25710=DIRECTION ( 'NONE',  ( 0.000000000000000000, 0.000000000000000000, 1.000000000000000000 ) ) ;
#25712=ORIENTED_EDGE ( 'NONE', *, *, #40603, .F. ) ;
#25713=AXIS2_PLACEMENT_3D ( 'NONE', #101198, #111663, #22011 ) ;
#25714=FACE_OUTER_BOUND ( 'NONE', #117038, .T. ) ;
#25716=EDGE_LOOP ( 'NONE', ( #30370, #72122, #42758, #22758 ) ) ;
#25718=LINE ( 'NONE', #95117, #129206 ) ;
#25719=DIRECTION ( 'NONE',  ( -0.000000000000000000, 1.000000000000000000, -0.000000000000000000 ) ) ;
#25720=CIRCLE ( 'NONE', #124016, 0.09999999999999982514 ) ;
#25721=ORIENTED_EDGE ( 'NONE', *, *, #34709, .F. ) ;
#25722=CARTESIAN_POINT ( 'NONE',  ( -10.65000000000000391, 2.500000000000000000, -6.741600689897074616 ) ) ;
#25723=ORIENTED_EDGE ( 'NONE', *, *, #126486, .F. ) ;
#25724=CARTESIAN_POINT ( 'NONE',  ( 0.4499999999999569344, 2.500000000000000000, 2.165063509461097713 ) ) ;
#25725=DIRECTION ( 'NONE',  ( 0.000000000000000000, 0.000000000000000000, 1.000000000000000000 ) ) ;
#25726=CONICAL_SURFACE ( 'NONE', #88417, 0.1000000000000000472, 0.003490658503988666988 ) ;
#25727=ORIENTED_EDGE ( 'NONE', *, *, #79414, .T. ) ;
#25728=CONICAL_SURFACE ( 'NONE', #67576, 0.09999999999999982514, 0.003490658503988666988 ) ;
#25729=ADVANCED_FACE ( 'NONE', ( #51699 ), #34418, .T. ) ;
#25730=AXIS2_PLACEMENT_3D ( 'NONE', #79238, #89050, #99526 ) ;
#25731=DIRECTION ( 'NONE',  ( 0.000000000000000000, -0.9999939076577903929, 0.003490651415223739937 ) ) ;
#25732=FACE_OUTER_BOUND ( 'NONE', #76129, .T. ) ;
#25733=ADVANCED_FACE ( 'NONE', ( #112555 ), #120432, .T. ) ;
#25734=AXIS2_PLACEMENT_3D ( 'NONE', #84505, #99798, #120087 ) ;
#25735=ADVANCED_FACE ( 'NONE', ( #32718 ), #121708, .T. ) ;
#25736=ORIENTED_EDGE ( 'NONE', *, *, #32348, .F. ) ;
#25737=VECTOR ( 'NONE', #41149, 1000.000000000000000 ) ;
#25738=LINE ( 'NONE', #65659, #26497 ) ;
#25739=CIRCLE ( 'NONE', #4796, 0.1000000000000000472 ) ;
#25740=AXIS2_PLACEMENT_3D ( 'NONE', #23784, #13942, #63056 ) ;
#25741=ORIENTED_EDGE ( 'NONE', *, *, #43845, .F. ) ;
#25742=VERTEX_POINT ( 'NONE', #91611 ) ;
#25743=CARTESIAN_POINT ( 'NONE',  ( -10.60000000000000142, 12.50000000000000000, 4.676537180435972552 ) ) ;
#25744=LINE ( 'NONE', #105610, #24930 ) ;
#25745=EDGE_CURVE ( 'NONE', #65132, #127833, #70000, .T. ) ;
#25746=EDGE_CURVE ( 'NONE', #68456, #58840, #60863, .T. ) ;
#25747=VERTEX_POINT ( 'NONE', #50393 ) ;
#25748=EDGE_CURVE ( 'NONE', #111170, #9181, #128510, .T. ) ;
#25749=DIRECTION ( 'NONE',  ( -0.000000000000000000, -1.000000000000000000, -0.000000000000000000 ) ) ;
#25750=CARTESIAN_POINT ( 'NONE',  ( -0.8000000000000376810, 12.50000000000000000, -4.395220292106239768 ) ) ;
#25751=AXIS2_PLACEMENT_3D ( 'NONE', #119588, #9648, #28658 ) ;
#25752=ORIENTED_EDGE ( 'NONE', *, *, #57138, .F. ) ;
#25753=DIRECTION ( 'NONE',  ( 0.000000000000000000, -0.000000000000000000, 1.000000000000000000 ) ) ;
#25754=CARTESIAN_POINT ( 'NONE',  ( 4.549999999999937650, 2.500000000000000000, 2.065063509461097624 ) ) ;
#25755=AXIS2_PLACEMENT_3D ( 'NONE', #10732, #57942, #97844 ) ;
#25756=CONICAL_SURFACE ( 'NONE', #6949, 0.09999999999999999167, 0.003490658503988666988 ) ;
#25757=AXIS2_PLACEMENT_3D ( 'NONE', #49004, #128197, #99385 ) ;
#25758=CARTESIAN_POINT ( 'NONE',  ( -4.600000000000025402, 12.50000000000000000, -2.385244779468109755E-15 ) ) ;
#25760=CARTESIAN_POINT ( 'NONE',  ( -12.94999999999999218, 2.500000000000000000, -2.065063509461099844 ) ) ;
#25761=AXIS2_PLACEMENT_3D ( 'NONE', #55392, #14782, #54729 ) ;
#25762=DIRECTION ( 'NONE',  ( 0.000000000000000000, 0.000000000000000000, -1.000000000000000000 ) ) ;
#25763=ORIENTED_EDGE ( 'NONE', *, *, #101964, .F. ) ;
#25764=CIRCLE ( 'NONE', #48768, 0.09999999999999982514 ) ;
#25765=ORIENTED_EDGE ( 'NONE', *, *, #111671, .F. ) ;
#25766=EDGE_LOOP ( 'NONE', ( #102469, #90224 ) ) ;
#25767=ORIENTED_EDGE ( 'NONE', *, *, #52100, .F. ) ;
#25768=DIRECTION ( 'NONE',  ( -0.000000000000000000, 1.000000000000000000, -0.000000000000000000 ) ) ;
#25769=DIRECTION ( 'NONE',  ( 0.000000000000000000, 0.000000000000000000, 1.000000000000000000 ) ) ;
#25770=CARTESIAN_POINT ( 'NONE',  ( 11.64999999999990798, 2.500000000000000000, 5.902370205355745192 ) ) ;
#25771=ORIENTED_EDGE ( 'NONE', *, *, #59049, .F. ) ;
#25772=FACE_BOUND ( 'NONE', #83413, .T. ) ;
#25773=DIRECTION ( 'NONE',  ( 0.000000000000000000, -0.000000000000000000, 1.000000000000000000 ) ) ;
#25774=CARTESIAN_POINT ( 'NONE',  ( 9.799999999999917222, 12.50000000000000000, 0.3464101615137735735 ) ) ;
#25775=PLANE ( 'NONE',  #59656 ) ;
#25776=PLANE ( 'NONE',  #53419 ) ;
#25777=DIRECTION ( 'NONE',  ( 0.000000000000000000, 1.000000000000000000, 0.000000000000000000 ) ) ;
#25778=CARTESIAN_POINT ( 'NONE',  ( -13.34999999999999076, 2.500000000000000000, -2.957883832488651610 ) ) ;
#25779=DIRECTION ( 'NONE',  ( -0.000000000000000000, -1.000000000000000000, -0.000000000000000000 ) ) ;
#25780=CARTESIAN_POINT ( 'NONE',  ( -3.150000000000030109, 12.50000000000000000, 1.818653347947321475 ) ) ;
#25781=CIRCLE ( 'NONE', #23740, 0.06509327318403745899 ) ;
#25782=CIRCLE ( 'NONE', #735, 0.1000000000000002554 ) ;
#25783=LINE ( 'NONE', #126573, #64111 ) ;
#25784=DIRECTION ( 'NONE',  ( 0.000000000000000000, 0.000000000000000000, -1.000000000000000000 ) ) ;
#25785=CIRCLE ( 'NONE', #9060, 7.500000000000000000 ) ;
#25786=EDGE_LOOP ( 'NONE', ( #52745, #98241, #75770, #63968 ) ) ;
#25787=ORIENTED_EDGE ( 'NONE', *, *, #41630, .F. ) ;
#25788=EDGE_LOOP ( 'NONE', ( #107932, #40914 ) ) ;
#25789=CONICAL_SURFACE ( 'NONE', #69705, 0.09999999999999999167, 0.003490658503988666988 ) ;
#25790=ORIENTED_EDGE ( 'NONE', *, *, #56724, .F. ) ;
#25791=CARTESIAN_POINT ( 'NONE',  ( -9.550000000000007816, 12.50000000000000000, -6.560283801567334372 ) ) ;
#25792=CONICAL_SURFACE ( 'NONE', #113621, 0.1000000000000002554, 0.003490658503988666988 ) ;
#25793=ORIENTED_EDGE ( 'NONE', *, *, #9634, .F. ) ;
#25794=CIRCLE ( 'NONE', #59266, 0.09999999999999982514 ) ;
#25795=ADVANCED_FACE ( 'NONE', ( #71986 ), #643, .T. ) ;
#25796=DIRECTION ( 'NONE',  ( 0.000000000000000000, 1.000000000000000000, 0.000000000000000000 ) ) ;
#25797=EDGE_CURVE ( 'NONE', #70661, #81572, #73259, .T. ) ;
#25798=EDGE_LOOP ( 'NONE', ( #107764, #42117 ) ) ;
#25799=VERTEX_POINT ( 'NONE', #81776 ) ;
#25800=EDGE_CURVE ( 'NONE', #26024, #48610, #111903, .T. ) ;
#25801=DIRECTION ( 'NONE',  ( -4.274815082592931898E-19, -0.9999939076577903929, -0.003490651415223739937 ) ) ;
#25802=AXIS2_PLACEMENT_3D ( 'NONE', #43917, #64821, #64179 ) ;
#25803=AXIS2_PLACEMENT_3D ( 'NONE', #40806, #89872, #30988 ) ;
#25804=AXIS2_PLACEMENT_3D ( 'NONE', #99763, #120045, #67704 ) ;
#25805=DIRECTION ( 'NONE',  ( 0.000000000000000000, -0.9999939076577903929, 0.003490651415223739937 ) ) ;
#25806=CARTESIAN_POINT ( 'NONE',  ( 8.549999999999920774, 2.500000000000000000, 6.148780366869520897 ) ) ;
#25807=LINE ( 'NONE', #53345, #101156 ) ;
#25808=EDGE_CURVE ( 'NONE', #79392, #72341, #62170, .T. ) ;
#25809=CARTESIAN_POINT ( 'NONE',  ( -5.000000000000026645, 2.500000000000000000, -3.737306695894649700 ) ) ;
#25810=CIRCLE ( 'NONE', #67547, 0.06509327318403745899 ) ;
#25811=ADVANCED_FACE ( 'NONE', ( #21583 ), #113818, .T. ) ;
#25812=ORIENTED_EDGE ( 'NONE', *, *, #10716, .T. ) ;
#25813=EDGE_CURVE ( 'NONE', #128257, #32927, #81158, .T. ) ;
#25814=EDGE_CURVE ( 'NONE', #17144, #2782, #72065, .T. ) ;
#25815=EDGE_LOOP ( 'NONE', ( #119977, #42147 ) ) ;
#25816=ADVANCED_FACE ( 'NONE', ( #52330 ), #84570, .T. ) ;
#25817=ORIENTED_EDGE ( 'NONE', *, *, #88142, .T. ) ;
#25819=DIRECTION ( 'NONE',  ( 0.000000000000000000, -0.000000000000000000, 1.000000000000000000 ) ) ;
#25820=ORIENTED_EDGE ( 'NONE', *, *, #5782, .T. ) ;
#25821=ORIENTED_EDGE ( 'NONE', *, *, #68680, .F. ) ;
#25822=ADVANCED_FACE ( 'NONE', ( #13026 ), #3240, .T. ) ;
#25823=AXIS2_PLACEMENT_3D ( 'NONE', #80645, #79985, #120559 ) ;
#25824=DIRECTION ( 'NONE',  ( -0.000000000000000000, -1.000000000000000000, -0.000000000000000000 ) ) ;
#25825=DIRECTION ( 'NONE',  ( 0.000000000000000000, 1.000000000000000000, 0.000000000000000000 ) ) ;
#25826=CARTESIAN_POINT ( 'NONE',  ( 10.84999999999990905, 2.500000000000000000, -6.595190528383302109 ) ) ;
#25828=CARTESIAN_POINT ( 'NONE',  ( -4.400000000000028777, 12.50000000000000000, -4.611443907251940644 ) ) ;
#25829=CARTESIAN_POINT ( 'NONE',  ( -11.64999999999999680, 12.50000000000000000, -7.253104124594887736 ) ) ;
#25830=VECTOR ( 'NONE', #33305, 1000.000000000000000 ) ;
#25831=ORIENTED_EDGE ( 'NONE', *, *, #7992, .T. ) ;
#25832=CARTESIAN_POINT ( 'NONE',  ( 4.999999999999969802, 2.500000000000000000, 4.430127018922196847 ) ) ;
#25833=CIRCLE ( 'NONE', #7022, 0.1000000000000002554 ) ;
#25834=VECTOR ( 'NONE', #123443, 1000.000000000000000 ) ;
#25835=ORIENTED_EDGE ( 'NONE', *, *, #100237, .F. ) ;
#25836=DIRECTION ( 'NONE',  ( -0.000000000000000000, -1.000000000000000000, -0.000000000000000000 ) ) ;
#25837=ORIENTED_EDGE ( 'NONE', *, *, #89150, .F. ) ;
#25838=PLANE ( 'NONE',  #118404 ) ;
#25839=DIRECTION ( 'NONE',  ( 0.000000000000000000, 0.000000000000000000, 1.000000000000000000 ) ) ;
#25841=EDGE_LOOP ( 'NONE', ( #81665, #81822, #110232, #60754 ) ) ;
#25842=DIRECTION ( 'NONE',  ( -0.000000000000000000, 1.000000000000000000, -0.000000000000000000 ) ) ;
#25843=DIRECTION ( 'NONE',  ( 0.000000000000000000, -0.9999939076577903929, 0.003490651415223739937 ) ) ;
#25844=AXIS2_PLACEMENT_3D ( 'NONE', #54247, #122990, #3849 ) ;
#25845=EDGE_LOOP ( 'NONE', ( #43217, #24510, #104370, #106616 ) ) ;
#25846=AXIS2_PLACEMENT_3D ( 'NONE', #27274, #107116, #27926 ) ;
#25847=VECTOR ( 'NONE', #116260, 1000.000000000000000 ) ;
#25848=DIRECTION ( 'NONE',  ( -0.000000000000000000, 1.000000000000000000, -0.000000000000000000 ) ) ;
#25849=CONICAL_SURFACE ( 'NONE', #21645, 0.1000000000000002554, 0.003490658503988666988 ) ;
#25850=CARTESIAN_POINT ( 'NONE',  ( 7.899999999999923084, 12.50000000000000000, 0.6928203230275494784 ) ) ;
#25851=ORIENTED_EDGE ( 'NONE', *, *, #57412, .T. ) ;
#25852=EDGE_LOOP ( 'NONE', ( #55668, #46008, #90553, #95466 ) ) ;
#25853=CARTESIAN_POINT ( 'NONE',  ( 10.64999999999990976, 12.50000000000000000, 2.511473670974873507 ) ) ;
#25856=VECTOR ( 'NONE', #14805, 1000.000000000000000 ) ;
#25857=DIRECTION ( 'NONE',  ( -0.000000000000000000, -1.000000000000000000, -0.000000000000000000 ) ) ;
#25858=CARTESIAN_POINT ( 'NONE',  ( -10.60000000000000142, 2.500000000000000000, 4.776537180435972196 ) ) ;
#25859=EDGE_CURVE ( 'NONE', #109438, #49236, #123013, .T. ) ;
#25860=AXIS2_PLACEMENT_3D ( 'NONE', #79234, #89686, #48474 ) ;
#25861=AXIS2_PLACEMENT_3D ( 'NONE', #25301, #83612, #54772 ) ;
#25862=DIRECTION ( 'NONE',  ( -4.274815082592931898E-19, -0.9999939076577903929, -0.003490651415223739937 ) ) ;
#25863=CIRCLE ( 'NONE', #107331, 0.09999999999999999167 ) ;
#25864=ORIENTED_EDGE ( 'NONE', *, *, #99936, .F. ) ;
#25865=CONICAL_SURFACE ( 'NONE', #73982, 0.1000000000000002554, 0.003490658503988666988 ) ;
#25866=CARTESIAN_POINT ( 'NONE',  ( 43.31345875132075918, 2.029331038885034744, -5.113051027236704016 ) ) ;
#25867=ORIENTED_EDGE ( 'NONE', *, *, #42941, .T. ) ;
#25868=ADVANCED_FACE ( 'NONE', ( #3871 ), #53624, .T. ) ;
#25869=CARTESIAN_POINT ( 'NONE',  ( 13.34999999999990017, 12.50000000000000000, 2.230156782645134950 ) ) ;
#25870=DIRECTION ( 'NONE',  ( 0.000000000000000000, 1.000000000000000000, 0.000000000000000000 ) ) ;
#25871=CARTESIAN_POINT ( 'NONE',  ( -4.400000000000025224, 12.50000000000000000, 4.676537180435972552 ) ) ;
#25872=VERTEX_POINT ( 'NONE', #116393 ) ;
#25873=DIRECTION ( 'NONE',  ( -0.000000000000000000, -1.000000000000000000, -0.000000000000000000 ) ) ;
#25874=DIRECTION ( 'NONE',  ( 0.000000000000000000, 0.000000000000000000, -1.000000000000000000 ) ) ;
#25875=AXIS2_PLACEMENT_3D ( 'NONE', #40504, #30680, #70581 ) ;
#25876=CIRCLE ( 'NONE', #13338, 0.09999999999999982514 ) ;
#25877=VERTEX_POINT ( 'NONE', #125567 ) ;
#25878=DIRECTION ( 'NONE',  ( -0.000000000000000000, -1.000000000000000000, -0.000000000000000000 ) ) ;
#25879=AXIS2_PLACEMENT_3D ( 'NONE', #86733, #46161, #57281 ) ;
#25880=VECTOR ( 'NONE', #28594, 1000.000000000000000 ) ;
#25881=ORIENTED_EDGE ( 'NONE', *, *, #16942, .T. ) ;
#25882=CIRCLE ( 'NONE', #96986, 0.1000000000000002554 ) ;
#25883=ORIENTED_EDGE ( 'NONE', *, *, #68527, .F. ) ;
#25884=DIRECTION ( 'NONE',  ( 0.000000000000000000, 1.000000000000000000, 0.000000000000000000 ) ) ;
#25885=CIRCLE ( 'NONE', #2907, 0.06509327318403745899 ) ;
#25886=AXIS2_PLACEMENT_3D ( 'NONE', #28272, #68180, #28929 ) ;
#25887=ORIENTED_EDGE ( 'NONE', *, *, #31431, .T. ) ;
#25888=DIRECTION ( 'NONE',  ( -4.274815082592931898E-19, -0.9999939076577903929, -0.003490651415223739937 ) ) ;
#25889=DIRECTION ( 'NONE',  ( 0.000000000000000000, 0.000000000000000000, 1.000000000000000000 ) ) ;
#25890=DIRECTION ( 'NONE',  ( 0.000000000000000000, 0.000000000000000000, 1.000000000000000000 ) ) ;
#25891=CIRCLE ( 'NONE', #78227, 0.1000000000000002554 ) ;
#25892=ORIENTED_EDGE ( 'NONE', *, *, #25982, .F. ) ;
#25893=AXIS2_PLACEMENT_3D ( 'NONE', #16311, #15670, #125000 ) ;
#25894=CONICAL_SURFACE ( 'NONE', #42646, 0.09999999999999999167, 0.003490658503988666988 ) ;
#25895=EDGE_CURVE ( 'NONE', #38108, #114128, #111759, .T. ) ;
#25896=FACE_BOUND ( 'NONE', #40108, .T. ) ;
#25897=DIRECTION ( 'NONE',  ( -0.000000000000000000, 1.000000000000000000, -0.000000000000000000 ) ) ;
#25898=VERTEX_POINT ( 'NONE', #36583 ) ;
#25899=CIRCLE ( 'NONE', #53089, 0.06509327318403745899 ) ;
#25900=LINE ( 'NONE', #75001, #500 ) ;
#25901=LINE ( 'NONE', #65809, #119919 ) ;
#25902=EDGE_CURVE ( 'NONE', #44383, #89842, #88776, .T. ) ;
#25903=EDGE_LOOP ( 'NONE', ( #22178, #74515, #64398, #1244 ) ) ;
#25904=EDGE_LOOP ( 'NONE', ( #88407, #28266 ) ) ;
#25905=ORIENTED_EDGE ( 'NONE', *, *, #66933, .F. ) ;
#25906=DIRECTION ( 'NONE',  ( -0.000000000000000000, -1.000000000000000000, -0.000000000000000000 ) ) ;
#25907=FACE_OUTER_BOUND ( 'NONE', #87911, .T. ) ;
#25908=EDGE_CURVE ( 'NONE', #60793, #7675, #118005, .T. ) ;
#25909=EDGE_CURVE ( 'NONE', #55580, #115142, #9349, .T. ) ;
#25910=DIRECTION ( 'NONE',  ( -0.000000000000000000, -1.000000000000000000, -0.000000000000000000 ) ) ;
#25911=EDGE_CURVE ( 'NONE', #58191, #22696, #78329, .T. ) ;
#25912=FACE_BOUND ( 'NONE', #34395, .T. ) ;
#25913=ORIENTED_EDGE ( 'NONE', *, *, #96139, .F. ) ;
#25914=EDGE_CURVE ( 'NONE', #105966, #63642, #13544, .T. ) ;
#25916=EDGE_CURVE ( 'NONE', #31579, #127574, #5137, .T. ) ;
#25917=CARTESIAN_POINT ( 'NONE',  ( -2.499999999999996003, 2.500000000000000000, 0.09999999999999772959 ) ) ;
#25919=AXIS2_PLACEMENT_3D ( 'NONE', #75960, #79207, #128963 ) ;
#25920=CARTESIAN_POINT ( 'NONE',  ( -3.750000000000026201, 12.50000000000000000, 5.802370205355744659 ) ) ;
#25921=LINE ( 'NONE', #55380, #71576 ) ;
#25922=PLANE ( 'NONE',  #115506 ) ;
#25923=EDGE_CURVE ( 'NONE', #33163, #90278, #97085, .T. ) ;
#25924=FACE_OUTER_BOUND ( 'NONE', #117770, .T. ) ;
#25925=CARTESIAN_POINT ( 'NONE',  ( -10.65000000000000213, 2.500000000000000000, 2.611473670974873151 ) ) ;
#25926=VECTOR ( 'NONE', #88876, 1000.000000000000000 ) ;
#25928=AXIS2_PLACEMENT_3D ( 'NONE', #117808, #56953, #35412 ) ;
#25929=EDGE_CURVE ( 'NONE', #44028, #4134, #124284, .T. ) ;
#25930=CARTESIAN_POINT ( 'NONE',  ( -3.750000000000025757, 12.50000000000000000, 1.407149913249508000 ) ) ;
#25931=ORIENTED_EDGE ( 'NONE', *, *, #15820, .T. ) ;
#25932=ORIENTED_EDGE ( 'NONE', *, *, #18717, .T. ) ;
#25933=VERTEX_POINT ( 'NONE', #56187 ) ;
#25934=ORIENTED_EDGE ( 'NONE', *, *, #128561, .F. ) ;
#25935=ORIENTED_EDGE ( 'NONE', *, *, #25320, .F. ) ;
#25936=LINE ( 'NONE', #6264, #379 ) ;
#25937=DIRECTION ( 'NONE',  ( 0.000000000000000000, -0.9999939076577903929, 0.003490651415223739937 ) ) ;
#25938=ORIENTED_EDGE ( 'NONE', *, *, #33960, .F. ) ;
#25939=FACE_BOUND ( 'NONE', #440, .T. ) ;
#25940=AXIS2_PLACEMENT_3D ( 'NONE', #12846, #41073, #31877 ) ;
#25941=DIRECTION ( 'NONE',  ( 0.000000000000000000, 1.000000000000000000, 0.000000000000000000 ) ) ;
#25942=VECTOR ( 'NONE', #129343, 1000.000000000000000 ) ;
#25943=CIRCLE ( 'NONE', #122091, 0.06509327318403745899 ) ;
#25944=CARTESIAN_POINT ( 'NONE',  ( -10.80000000000000249, 12.50000000000000000, -4.330127018922197202 ) ) ;
#25945=LINE ( 'NONE', #56661, #11884 ) ;
#25946=CARTESIAN_POINT ( 'NONE',  ( -6.900000000000019007, 12.50000000000000000, -0.2813168883297409439 ) ) ;
#25947=PLANE ( 'NONE',  #89358 ) ;
#25948=ORIENTED_EDGE ( 'NONE', *, *, #15334, .F. ) ;
#25949=DIRECTION ( 'NONE',  ( -4.274815082592931898E-19, -0.9999939076577903929, -0.003490651415223739937 ) ) ;
#25950=EDGE_LOOP ( 'NONE', ( #100604, #70337 ) ) ;
#25951=CIRCLE ( 'NONE', #13413, 0.06509327318403745899 ) ;
#25953=ORIENTED_EDGE ( 'NONE', *, *, #128507, .T. ) ;
#25954=DIRECTION ( 'NONE',  ( 0.000000000000000000, 0.000000000000000000, 1.000000000000000000 ) ) ;
#25955=PLANE ( 'NONE',  #64436 ) ;
#25956=CARTESIAN_POINT ( 'NONE',  ( 1.449999999999952216, 2.500000000000000000, -2.611473670974877592 ) ) ;
#25957=AXIS2_PLACEMENT_3D ( 'NONE', #37540, #58476, #108830 ) ;
#25958=ORIENTED_EDGE ( 'NONE', *, *, #87960, .T. ) ;
#25959=CARTESIAN_POINT ( 'NONE',  ( 16.04820284657640173, 2.500000000000064393, -6.585610460626884155 ) ) ;
#25960=EDGE_CURVE ( 'NONE', #57754, #117365, #83732, .T. ) ;
#25961=AXIS2_PLACEMENT_3D ( 'NONE', #37819, #107195, #17520 ) ;
#25962=CARTESIAN_POINT ( 'NONE',  ( 10.64999999999990976, 2.500000000000000000, 2.511473670974873507 ) ) ;
#25963=EDGE_CURVE ( 'NONE', #39201, #90179, #80376, .T. ) ;
#25964=CARTESIAN_POINT ( 'NONE',  ( 6.649999999999928413, 2.500000000000000000, 1.472243186433545459 ) ) ;
#25966=DIRECTION ( 'NONE',  ( -0.000000000000000000, -1.000000000000000000, -0.000000000000000000 ) ) ;
#25967=LINE ( 'NONE', #37081, #39147 ) ;
#25968=EDGE_CURVE ( 'NONE', #112183, #44934, #75827, .T. ) ;
#25969=ORIENTED_EDGE ( 'NONE', *, *, #67033, .F. ) ;
#25970=CARTESIAN_POINT ( 'NONE',  ( 5.399999999999932854, 12.50000000000000000, 5.022947341949748790 ) ) ;
#25971=ADVANCED_FACE ( 'NONE', ( #104014 ), #45742, .T. ) ;
#25972=ORIENTED_EDGE ( 'NONE', *, *, #50853, .T. ) ;
#25973=ADVANCED_FACE ( 'NONE', ( #123632 ), #32374, .T. ) ;
#25974=ORIENTED_EDGE ( 'NONE', *, *, #48535, .T. ) ;
#25975=FACE_OUTER_BOUND ( 'NONE', #40821, .T. ) ;
#25976=AXIS2_PLACEMENT_3D ( 'NONE', #11670, #63997, #22807 ) ;
#25977=CONICAL_SURFACE ( 'NONE', #128402, 0.1000000000000002554, 0.003490658503988666988 ) ;
#25978=CARTESIAN_POINT ( 'NONE',  ( -8.550000000000013145, 12.50000000000000000, 2.446380397790835826 ) ) ;
#25979=CONICAL_SURFACE ( 'NONE', #42727, 0.1000000000000002554, 0.003490658503988666988 ) ;
#25980=CARTESIAN_POINT ( 'NONE',  ( 0.1999999999999576006, 2.500000000000000000, -4.676537180435978769 ) ) ;
#25981=VERTEX_POINT ( 'NONE', #114468 ) ;
#25982=EDGE_CURVE ( 'NONE', #85528, #80364, #99253, .T. ) ;
#25983=EDGE_LOOP ( 'NONE', ( #96593, #94912 ) ) ;
#25984=DIRECTION ( 'NONE',  ( 0.000000000000000000, 1.000000000000000000, 0.000000000000000000 ) ) ;
#25986=AXIS2_PLACEMENT_3D ( 'NONE', #6334, #46283, #126139 ) ;
#25987=VECTOR ( 'NONE', #40984, 1000.000000000000000 ) ;
#25988=CARTESIAN_POINT ( 'NONE',  ( 8.749999999999920064, 2.500000000000000000, 5.802370205355744659 ) ) ;
#25989=AXIS2_PLACEMENT_3D ( 'NONE', #112277, #52065, #62534 ) ;
#25990=CARTESIAN_POINT ( 'NONE',  ( -3.950000000000026379, 2.500000000000000000, 6.741600689897071952 ) ) ;
#25991=ORIENTED_EDGE ( 'NONE', *, *, #49032, .T. ) ;
#25992=VERTEX_POINT ( 'NONE', #65359 ) ;
#25993=CARTESIAN_POINT ( 'NONE',  ( 13.54999999999989591, 2.500000000000000000, -1.718653347947326049 ) ) ;
#25994=ORIENTED_EDGE ( 'NONE', *, *, #66567, .F. ) ;
#25995=DIRECTION ( 'NONE',  ( 0.000000000000000000, 0.000000000000000000, -1.000000000000000000 ) ) ;
#25996=CIRCLE ( 'NONE', #13450, 0.1000000000000002554 ) ;
#25997=CONICAL_SURFACE ( 'NONE', #65685, 0.09999999999999982514, 0.003490658503988666988 ) ;
#25998=DIRECTION ( 'NONE',  ( -0.000000000000000000, -1.000000000000000000, -0.000000000000000000 ) ) ;
#25999=VERTEX_POINT ( 'NONE', #57495 ) ;
#26000=CARTESIAN_POINT ( 'NONE',  ( -9.350000000000006750, 12.50000000000000000, 2.576566944158910744 ) ) ;
#26001=DIRECTION ( 'NONE',  ( 0.000000000000000000, 1.000000000000000000, 0.000000000000000000 ) ) ;
#26002=DIRECTION ( 'NONE',  ( 0.000000000000000000, 1.000000000000000000, 0.000000000000000000 ) ) ;
#26003=VECTOR ( 'NONE', #110523, 1000.000000000000000 ) ;
#26004=EDGE_CURVE ( 'NONE', #107927, #79022, #59563, .T. ) ;
#26005=CARTESIAN_POINT ( 'NONE',  ( 1.899999999999949507, 2.500000000000000000, 3.983716857408420964 ) ) ;
#26006=ORIENTED_EDGE ( 'NONE', *, *, #60912, .T. ) ;
#26007=CARTESIAN_POINT ( 'NONE',  ( -11.44999999999999751, 2.500000000000000000, 1.718653347947321386 ) ) ;
#26008=DIRECTION ( 'NONE',  ( -4.274815082592931898E-19, -0.9999939076577903929, -0.003490651415223739937 ) ) ;
#26009=ORIENTED_EDGE ( 'NONE', *, *, #42330, .T. ) ;
#26010=VERTEX_POINT ( 'NONE', #41580 ) ;
#26012=CARTESIAN_POINT ( 'NONE',  ( -7.100000000000017408, 2.500000000000000000, -3.637306695894650055 ) ) ;
#26013=DIRECTION ( 'NONE',  ( 0.000000000000000000, 1.000000000000000000, 0.000000000000000000 ) ) ;
#26014=CARTESIAN_POINT ( 'NONE',  ( -2.900000000000029221, 2.500000000000000000, -5.022947341949754119 ) ) ;
#26015=VECTOR ( 'NONE', #125691, 1000.000000000000000 ) ;
#26016=LINE ( 'NONE', #37760, #926 ) ;
#26017=DIRECTION ( 'NONE',  ( 0.000000000000000000, 0.000000000000000000, 1.000000000000000000 ) ) ;
#26018=DIRECTION ( 'NONE',  ( 0.000000000000000000, 1.000000000000000000, 0.000000000000000000 ) ) ;
#26019=EDGE_CURVE ( 'NONE', #60793, #21571, #110292, .T. ) ;
#26020=DIRECTION ( 'NONE',  ( 0.000000000000000000, -0.000000000000000000, 1.000000000000000000 ) ) ;
#26021=DIRECTION ( 'NONE',  ( 0.000000000000000000, 1.000000000000000000, 0.000000000000000000 ) ) ;
#26022=DIRECTION ( 'NONE',  ( 0.000000000000000000, -0.000000000000000000, 1.000000000000000000 ) ) ;
#26023=CONICAL_SURFACE ( 'NONE', #34438, 0.1000000000000000472, 0.003490658503988666988 ) ;
#26024=VERTEX_POINT ( 'NONE', #117025 ) ;
#26025=CONICAL_SURFACE ( 'NONE', #34440, 0.1000000000000002554, 0.003490658503988666988 ) ;
#26026=VERTEX_POINT ( 'NONE', #28032 ) ;
#26027=ORIENTED_EDGE ( 'NONE', *, *, #33172, .T. ) ;
#26028=EDGE_CURVE ( 'NONE', #94609, #124362, #73087, .T. ) ;
#26029=DIRECTION ( 'NONE',  ( 0.000000000000000000, 0.000000000000000000, 1.000000000000000000 ) ) ;
#26030=DIRECTION ( 'NONE',  ( 0.000000000000000000, -0.000000000000000000, 1.000000000000000000 ) ) ;
#26031=CARTESIAN_POINT ( 'NONE',  ( -11.05000000000000249, 12.50000000000000000, -1.753560074763284682 ) ) ;
#26032=VERTEX_POINT ( 'NONE', #77130 ) ;
#26033=CARTESIAN_POINT ( 'NONE',  ( -2.499999999999996003, 2.500000000000000000, -0.1000000000000022815 ) ) ;
#26034=AXIS2_PLACEMENT_3D ( 'NONE', #70322, #49408, #89313 ) ;
#26035=AXIS2_PLACEMENT_3D ( 'NONE', #35437, #75337, #115234 ) ;
#26036=CARTESIAN_POINT ( 'NONE',  ( -14.59999999999998366, 12.50000000000000000, -1.084202172485504434E-16 ) ) ;
#26037=VERTEX_POINT ( 'NONE', #81485 ) ;
#26038=DIRECTION ( 'NONE',  ( 0.000000000000000000, 0.000000000000000000, -1.000000000000000000 ) ) ;
#26039=ORIENTED_EDGE ( 'NONE', *, *, #118236, .F. ) ;
#26040=AXIS2_PLACEMENT_3D ( 'NONE', #41378, #112684, #31542 ) ;
#26041=AXIS2_PLACEMENT_3D ( 'NONE', #108356, #9521, #27869 ) ;
#26042=ORIENTED_EDGE ( 'NONE', *, *, #49644, .T. ) ;
#26043=EDGE_LOOP ( 'NONE', ( #11044, #6468, #91181, #127283 ) ) ;
#26044=ORIENTED_EDGE ( 'NONE', *, *, #78274, .F. ) ;
#26045=DIRECTION ( 'NONE',  ( -0.000000000000000000, 1.000000000000000000, -0.000000000000000000 ) ) ;
#26046=CIRCLE ( 'NONE', #88738, 0.09999999999999982514 ) ;
#26047=CARTESIAN_POINT ( 'NONE',  ( 0.8499999999999550138, 12.50000000000000000, -5.802370205355749988 ) ) ;
#26048=CARTESIAN_POINT ( 'NONE',  ( 2.899999999999943956, 12.50000000000000000, 4.330127018922196314 ) ) ;
#26049=CIRCLE ( 'NONE', #46986, 0.06509327318403745899 ) ;
#26050=CARTESIAN_POINT ( 'NONE',  ( 5.199999999999933564, 2.500000000000000000, 0.3464101615137735735 ) ) ;
#26051=EDGE_LOOP ( 'NONE', ( #31125, #126761 ) ) ;
#26052=EDGE_CURVE ( 'NONE', #15482, #90797, #92987, .T. ) ;
#26053=DIRECTION ( 'NONE',  ( 0.000000000000000000, 0.000000000000000000, -1.000000000000000000 ) ) ;
#26054=EDGE_LOOP ( 'NONE', ( #8652, #125730 ) ) ;
#26055=CARTESIAN_POINT ( 'NONE',  ( 7.099999999999928590, 2.500000000000000000, 4.230127018922196669 ) ) ;
#26056=CARTESIAN_POINT ( 'NONE',  ( 13.80955901367097916, -1.500000000000063061, -7.955427458311421063 ) ) ;
#26057=DIRECTION ( 'NONE',  ( -4.274815082592931898E-19, -0.9999939076577903929, -0.003490651415223739937 ) ) ;
#26058=CARTESIAN_POINT ( 'NONE',  ( 16.79927703354229607, -2.472530191752539075, 3.248144252804014975 ) ) ;
#26059=EDGE_CURVE ( 'NONE', #1993, #61083, #88862, .T. ) ;
#26060=ORIENTED_EDGE ( 'NONE', *, *, #128758, .T. ) ;
#26061=AXIS2_PLACEMENT_3D ( 'NONE', #9094, #39239, #11013 ) ;
#26062=ORIENTED_EDGE ( 'NONE', *, *, #82971, .T. ) ;
#26063=AXIS2_PLACEMENT_3D ( 'NONE', #119529, #10848, #108424 ) ;
#26064=ORIENTED_EDGE ( 'NONE', *, *, #124397, .T. ) ;
#26065=DIRECTION ( 'NONE',  ( 0.000000000000000000, -0.9999939076577903929, 0.003490651415223739937 ) ) ;
#26067=EDGE_CURVE ( 'NONE', #101516, #116590, #80845, .T. ) ;
#26069=CARTESIAN_POINT ( 'NONE',  ( 11.84999999999990727, 12.50000000000000000, 6.148780366869520009 ) ) ;
#26071=FACE_BOUND ( 'NONE', #122450, .T. ) ;
#26072=ADVANCED_FACE ( 'NONE', ( #100472 ), #9452, .T. ) ;
#26073=LINE ( 'NONE', #105919, #116264 ) ;
#26074=CARTESIAN_POINT ( 'NONE',  ( 11.24999999999990941, 12.50000000000000000, -1.472243186433550122 ) ) ;
#26075=LINE ( 'NONE', #52453, #43469 ) ;
#26077=AXIS2_PLACEMENT_3D ( 'NONE', #19006, #30153, #50414 ) ;
#26078=AXIS2_PLACEMENT_3D ( 'NONE', #50006, #17937, #29072 ) ;
#26081=AXIS2_PLACEMENT_3D ( 'NONE', #41188, #12333, #81097 ) ;
#26082=EDGE_CURVE ( 'NONE', #119417, #29857, #60574, .T. ) ;
#26084=EDGE_CURVE ( 'NONE', #16737, #29270, #101121, .T. ) ;
#26085=DIRECTION ( 'NONE',  ( 0.000000000000000000, 1.000000000000000000, 0.000000000000000000 ) ) ;
#26086=EDGE_CURVE ( 'NONE', #108562, #30880, #21988, .T. ) ;
#26087=AXIS2_PLACEMENT_3D ( 'NONE', #116298, #86849, #26651 ) ;
#26088=AXIS2_PLACEMENT_3D ( 'NONE', #14320, #126228, #96115 ) ;
#26089=EDGE_CURVE ( 'NONE', #32323, #112846, #90921, .T. ) ;
#26090=DIRECTION ( 'NONE',  ( 0.000000000000000000, 1.000000000000000000, 0.000000000000000000 ) ) ;
#26091=ORIENTED_EDGE ( 'NONE', *, *, #50618, .T. ) ;
#26092=ORIENTED_EDGE ( 'NONE', *, *, #63674, .T. ) ;
#26093=VERTEX_POINT ( 'NONE', #117665 ) ;
#26094=VERTEX_POINT ( 'NONE', #58148 ) ;
#26095=AXIS2_PLACEMENT_3D ( 'NONE', #128753, #110367, #29251 ) ;
#26097=FACE_BOUND ( 'NONE', #24302, .T. ) ;
#26099=DIRECTION ( 'NONE',  ( -0.000000000000000000, -1.000000000000000000, -0.000000000000000000 ) ) ;
#26100=ORIENTED_EDGE ( 'NONE', *, *, #109419, .F. ) ;
#26101=CARTESIAN_POINT ( 'NONE',  ( 48.84100846696811971, 2.320798421900499342, 5.300800859553110200 ) ) ;
#26102=DIRECTION ( 'NONE',  ( -0.000000000000000000, -1.000000000000000000, -0.000000000000000000 ) ) ;
#26103=CIRCLE ( 'NONE', #7202, 0.1000000000000000472 ) ;
#26104=ORIENTED_EDGE ( 'NONE', *, *, #124792, .F. ) ;
#26105=DIRECTION ( 'NONE',  ( 0.000000000000000000, 1.000000000000000000, 0.000000000000000000 ) ) ;
#26106=CARTESIAN_POINT ( 'NONE',  ( -3.350000000000031619, 2.500000000000000000, -5.802370205355749988 ) ) ;
#26107=ORIENTED_EDGE ( 'NONE', *, *, #48364, .F. ) ;
#26108=CARTESIAN_POINT ( 'NONE',  ( 1.049999999999953637, 2.500000000000000000, -1.918653347947326004 ) ) ;
#26109=LINE ( 'NONE', #106586, #120687 ) ;
#26110=CIRCLE ( 'NONE', #93015, 0.06509327318403745899 ) ;
#26111=ORIENTED_EDGE ( 'NONE', *, *, #110713, .F. ) ;
#26112=DIRECTION ( 'NONE',  ( -0.000000000000000000, 1.000000000000000000, -0.000000000000000000 ) ) ;
#26113=DIRECTION ( 'NONE',  ( 0.000000000000000000, 0.000000000000000000, 1.000000000000000000 ) ) ;
#26114=ORIENTED_EDGE ( 'NONE', *, *, #28757, .F. ) ;
#26115=FACE_OUTER_BOUND ( 'NONE', #27807, .T. ) ;
#26116=ORIENTED_EDGE ( 'NONE', *, *, #114199, .F. ) ;
#26117=ORIENTED_EDGE ( 'NONE', *, *, #69841, .F. ) ;
#26119=ORIENTED_EDGE ( 'NONE', *, *, #44596, .F. ) ;
#26120=DIRECTION ( 'NONE',  ( 0.000000000000000000, 1.000000000000000000, 0.000000000000000000 ) ) ;
#26121=FACE_OUTER_BOUND ( 'NONE', #127393, .T. ) ;
#26122=VECTOR ( 'NONE', #105583, 1000.000000000000000 ) ;
#26123=EDGE_CURVE ( 'NONE', #124197, #52455, #120121, .T. ) ;
#26124=VERTEX_POINT ( 'NONE', #30468 ) ;
#26125=AXIS2_PLACEMENT_3D ( 'NONE', #54270, #4488, #34654 ) ;
#26126=CARTESIAN_POINT ( 'NONE',  ( -11.44999999999999751, 12.50000000000000000, 6.083687093685483660 ) ) ;
#26127=EDGE_CURVE ( 'NONE', #55439, #23160, #37218, .T. ) ;
#26128=DIRECTION ( 'NONE',  ( -0.000000000000000000, 1.000000000000000000, -0.000000000000000000 ) ) ;
#26129=LINE ( 'NONE', #124324, #73710 ) ;
#26130=CARTESIAN_POINT ( 'NONE',  ( 8.299999999999922551, 12.50000000000000000, -4.265033745738164406 ) ) ;
#26131=CARTESIAN_POINT ( 'NONE',  ( 8.549999999999922551, 2.500000000000000000, 2.411473670974873862 ) ) ;
#26132=DIRECTION ( 'NONE',  ( -0.000000000000000000, 1.000000000000000000, -0.000000000000000000 ) ) ;
#26133=EDGE_CURVE ( 'NONE', #64399, #79354, #107653, .T. ) ;
#26134=EDGE_LOOP ( 'NONE', ( #29702, #113102, #52227, #24506 ) ) ;
#26136=CARTESIAN_POINT ( 'NONE',  ( -0.4000000000000331624, 12.50000000000000000, -0.6928203230275519209 ) ) ;
#26137=CIRCLE ( 'NONE', #5181, 0.1000000000000002554 ) ;
#26138=AXIS2_PLACEMENT_3D ( 'NONE', #33049, #72957, #112880 ) ;
#26139=CARTESIAN_POINT ( 'NONE',  ( 0.8499999999999553468, 12.50000000000000000, 1.407149913249508000 ) ) ;
#26140=DIRECTION ( 'NONE',  ( 0.000000000000000000, 1.000000000000000000, 0.000000000000000000 ) ) ;
#26141=ORIENTED_EDGE ( 'NONE', *, *, #43805, .T. ) ;
#26142=VERTEX_POINT ( 'NONE', #73576 ) ;
#26143=ORIENTED_EDGE ( 'NONE', *, *, #106779, .F. ) ;
#26144=FACE_OUTER_BOUND ( 'NONE', #125156, .T. ) ;
#26145=DIRECTION ( 'NONE',  ( 0.000000000000000000, 0.000000000000000000, -1.000000000000000000 ) ) ;
#26146=DIRECTION ( 'NONE',  ( 0.000000000000000000, 0.000000000000000000, 1.000000000000000000 ) ) ;
#26148=DIRECTION ( 'NONE',  ( 0.000000000000000000, -0.9999939076577903929, 0.003490651415223739937 ) ) ;
#26149=CARTESIAN_POINT ( 'NONE',  ( -14.54999999999998472, 2.500000000000000000, -2.165063509461099489 ) ) ;
#26150=DIRECTION ( 'NONE',  ( 0.000000000000000000, 0.000000000000000000, -1.000000000000000000 ) ) ;
#26151=DIRECTION ( 'NONE',  ( 0.000000000000000000, 1.000000000000000000, 0.000000000000000000 ) ) ;
#26152=CARTESIAN_POINT ( 'NONE',  ( 9.149999999999915090, 2.500000000000000000, -2.065063509461102065 ) ) ;
#26153=CIRCLE ( 'NONE', #45032, 0.06509327318403745899 ) ;
#26154=DIRECTION ( 'NONE',  ( -0.000000000000000000, -1.000000000000000000, -0.000000000000000000 ) ) ;
#26155=ORIENTED_EDGE ( 'NONE', *, *, #31142, .T. ) ;
#26156=CIRCLE ( 'NONE', #99313, 0.06509327318403745899 ) ;
#26157=AXIS2_PLACEMENT_3D ( 'NONE', #86704, #114236, #35680 ) ;
#26158=DIRECTION ( 'NONE',  ( 0.000000000000000000, 0.000000000000000000, 1.000000000000000000 ) ) ;
#26159=AXIS2_PLACEMENT_3D ( 'NONE', #93107, #122564, #42065 ) ;
#26160=VERTEX_POINT ( 'NONE', #44790 ) ;
#26161=VERTEX_POINT ( 'NONE', #84043 ) ;
#26162=CARTESIAN_POINT ( 'NONE',  ( -11.89999999999999680, 2.500000000000000000, 0.3464101615137776813 ) ) ;
#26163=DIRECTION ( 'NONE',  ( -4.274815082592931898E-19, -0.9999939076577903929, -0.003490651415223739937 ) ) ;
#26164=CARTESIAN_POINT ( 'NONE',  ( 11.64999999999990443, 2.500000000000000000, 2.857883832488649301 ) ) ;
#26165=DIRECTION ( 'NONE',  ( 0.000000000000000000, 1.000000000000000000, 0.000000000000000000 ) ) ;
#26166=CIRCLE ( 'NONE', #44949, 0.06509327318403745899 ) ;
#26167=DIRECTION ( 'NONE',  ( 0.000000000000000000, -0.9999939076577903929, 0.003490651415223739937 ) ) ;
#26168=DIRECTION ( 'NONE',  ( -0.000000000000000000, -1.000000000000000000, -0.000000000000000000 ) ) ;
#26169=FACE_OUTER_BOUND ( 'NONE', #37087, .T. ) ;
#26170=VERTEX_POINT ( 'NONE', #84698 ) ;
#26173=CARTESIAN_POINT ( 'NONE',  ( -3.749999999999991118, 12.50000000000000000, 2.099970236277060032 ) ) ;
#26174=AXIS2_PLACEMENT_3D ( 'NONE', #89433, #91365, #110984 ) ;
#26175=EDGE_LOOP ( 'NONE', ( #114180, #72064, #58522, #75633 ) ) ;
#26176=AXIS2_PLACEMENT_3D ( 'NONE', #64411, #2930, #23859 ) ;
#26177=ORIENTED_EDGE ( 'NONE', *, *, #67271, .F. ) ;
#26178=ORIENTED_EDGE ( 'NONE', *, *, #107038, .T. ) ;
#26179=VECTOR ( 'NONE', #26348, 1000.000000000000000 ) ;
#26180=EDGE_CURVE ( 'NONE', #86483, #117851, #12719, .T. ) ;
#26181=ADVANCED_FACE ( 'NONE', ( #33046 ), #38725, .T. ) ;
#26182=VERTEX_POINT ( 'NONE', #92591 ) ;
#26183=DIRECTION ( 'NONE',  ( 0.000000000000000000, 0.000000000000000000, 1.000000000000000000 ) ) ;
#26184=FACE_OUTER_BOUND ( 'NONE', #19331, .T. ) ;
#26185=DIRECTION ( 'NONE',  ( 0.000000000000000000, 0.000000000000000000, 1.000000000000000000 ) ) ;
#26186=CARTESIAN_POINT ( 'NONE',  ( -5.650000000000023448, 2.500000000000000000, -6.941600689897078347 ) ) ;
#26187=B_SPLINE_CURVE_WITH_KNOTS ( 'NONE', 3,
 ( #19562, #7798, #88950, #98113, #99428, #18267 ),
 .UNSPECIFIED., .F., .F.,
 ( 4, 2, 4 ),
 ( 0.000000000000000000, 0.5000000000000000000, 1.000000000000000000 ),
 .UNSPECIFIED. ) ;
#26188=DIRECTION ( 'NONE',  ( 0.000000000000000000, -0.9999939076577903929, 0.003490651415223739937 ) ) ;
#26189=ORIENTED_EDGE ( 'NONE', *, *, #77034, .T. ) ;
#26190=EDGE_CURVE ( 'NONE', #46899, #122246, #49182, .T. ) ;
#26191=PLANE ( 'NONE',  #114169 ) ;
#26192=CIRCLE ( 'NONE', #101412, 7.500000000000000000 ) ;
#26193=LINE ( 'NONE', #106672, #85364 ) ;
#26194=ORIENTED_EDGE ( 'NONE', *, *, #37299, .F. ) ;
#26195=ORIENTED_EDGE ( 'NONE', *, *, #125840, .T. ) ;
#26196=ORIENTED_EDGE ( 'NONE', *, *, #89631, .F. ) ;
#26197=DIRECTION ( 'NONE',  ( -0.000000000000000000, -1.000000000000000000, -0.000000000000000000 ) ) ;
#26198=CIRCLE ( 'NONE', #24144, 0.09999999999999982514 ) ;
#26199=AXIS2_PLACEMENT_3D ( 'NONE', #35616, #75516, #125903 ) ;
#26200=DIRECTION ( 'NONE',  ( -4.274815082592931898E-19, -0.9999939076577903929, -0.003490651415223739937 ) ) ;
#26201=DIRECTION ( 'NONE',  ( -0.000000000000000000, -1.000000000000000000, -0.000000000000000000 ) ) ;
#26202=AXIS2_PLACEMENT_3D ( 'NONE', #109642, #8839, #19306 ) ;
#26203=EDGE_LOOP ( 'NONE', ( #65106, #106674, #118992, #15326 ) ) ;
#26204=FACE_OUTER_BOUND ( 'NONE', #68119, .T. ) ;
#26205=CARTESIAN_POINT ( 'NONE',  ( 7.499999999999925393, 2.500000000000000000, 5.122947341949749323 ) ) ;
#26206=LINE ( 'NONE', #87690, #119408 ) ;
#26207=DIRECTION ( 'NONE',  ( -0.000000000000000000, -1.000000000000000000, -0.000000000000000000 ) ) ;
#26208=CARTESIAN_POINT ( 'NONE',  ( -3.350000000000028955, 12.50000000000000000, -2.230156782645139391 ) ) ;
#26209=AXIS2_PLACEMENT_3D ( 'NONE', #113954, #72106, #14441 ) ;
#26210=ADVANCED_FACE ( 'NONE', ( #52656 ), #28234, .T. ) ;
#26211=EDGE_LOOP ( 'NONE', ( #46104, #23469, #7188, #36208 ) ) ;
#26212=CARTESIAN_POINT ( 'NONE',  ( 11.04999999999990834, 2.500000000000000000, 1.818653347947321475 ) ) ;
#26213=AXIS2_PLACEMENT_3D ( 'NONE', #65858, #33206, #14797 ) ;
#26214=ORIENTED_EDGE ( 'NONE', *, *, #44376, .T. ) ;
#26215=ORIENTED_EDGE ( 'NONE', *, *, #84449, .T. ) ;
#26216=EDGE_CURVE ( 'NONE', #81046, #103611, #126523, .T. ) ;
#26217=ORIENTED_EDGE ( 'NONE', *, *, #56637, .T. ) ;
#26218=ADVANCED_FACE ( 'NONE', ( #74239 ), #44960, .T. ) ;
#26219=DIRECTION ( 'NONE',  ( 0.000000000000000000, 0.000000000000000000, 1.000000000000000000 ) ) ;
#26220=EDGE_CURVE ( 'NONE', #118224, #46019, #104342, .T. ) ;
#26221=FACE_BOUND ( 'NONE', #107634, .T. ) ;
#26222=EDGE_CURVE ( 'NONE', #106042, #101934, #120171, .T. ) ;
#26223=FACE_OUTER_BOUND ( 'NONE', #111516, .T. ) ;
#26224=LINE ( 'NONE', #67394, #73674 ) ;
#26225=CARTESIAN_POINT ( 'NONE',  ( 3.749999999999942268, 2.500000000000000000, -1.472243186433550122 ) ) ;
#26226=CIRCLE ( 'NONE', #65922, 0.06509327318403745899 ) ;
#26227=VECTOR ( 'NONE', #104344, 1000.000000000000000 ) ;
#26228=ADVANCED_FACE ( 'NONE', ( #124627 ), #62504, .T. ) ;
#26229=ORIENTED_EDGE ( 'NONE', *, *, #57386, .F. ) ;
#26230=FACE_OUTER_BOUND ( 'NONE', #78502, .T. ) ;
#26231=CARTESIAN_POINT ( 'NONE',  ( -7.950000000000012612, 2.500000000000000000, 2.065063509461097624 ) ) ;
#26232=EDGE_CURVE ( 'NONE', #126222, #92046, #19922, .T. ) ;
#26233=DIRECTION ( 'NONE',  ( -0.000000000000000000, 1.000000000000000000, -0.000000000000000000 ) ) ;
#26234=DIRECTION ( 'NONE',  ( 0.000000000000000000, -0.000000000000000000, 1.000000000000000000 ) ) ;
#26235=ORIENTED_EDGE ( 'NONE', *, *, #49500, .T. ) ;
#26236=DIRECTION ( 'NONE',  ( -0.000000000000000000, 1.000000000000000000, -0.000000000000000000 ) ) ;
#26237=EDGE_CURVE ( 'NONE', #18715, #95681, #103537, .T. ) ;
#26238=DIRECTION ( 'NONE',  ( -0.000000000000000000, -1.000000000000000000, -0.000000000000000000 ) ) ;
#26239=AXIS2_PLACEMENT_3D ( 'NONE', #109840, #60741, #89549 ) ;
#26240=ORIENTED_EDGE ( 'NONE', *, *, #14862, .T. ) ;
#26241=FACE_OUTER_BOUND ( 'NONE', #14272, .T. ) ;
#26242=EDGE_CURVE ( 'NONE', #108236, #50883, #101393, .T. ) ;
#26243=VECTOR ( 'NONE', #98100, 1000.000000000000000 ) ;
#26244=FACE_BOUND ( 'NONE', #4216, .T. ) ;
#26245=EDGE_CURVE ( 'NONE', #47855, #74712, #122060, .T. ) ;
#26246=CARTESIAN_POINT ( 'NONE',  ( 0.3999999999999568345, 12.50000000000000000, -4.957854068765716882 ) ) ;
#26247=AXIS2_PLACEMENT_3D ( 'NONE', #5479, #85347, #3564 ) ;
#26248=ORIENTED_EDGE ( 'NONE', *, *, #25468, .F. ) ;
#26249=DIRECTION ( 'NONE',  ( -0.000000000000000000, -1.000000000000000000, -0.000000000000000000 ) ) ;
#26250=CARTESIAN_POINT ( 'NONE',  ( 1.649999999999951061, 2.500000000000000000, -6.495190528383302464 ) ) ;
#26251=AXIS2_PLACEMENT_3D ( 'NONE', #34252, #116005, #26355 ) ;
#26252=ORIENTED_EDGE ( 'NONE', *, *, #81441, .T. ) ;
#26253=ORIENTED_EDGE ( 'NONE', *, *, #37788, .T. ) ;
#26255=ORIENTED_EDGE ( 'NONE', *, *, #79539, .T. ) ;
#26257=CARTESIAN_POINT ( 'NONE',  ( -6.450000000000014388, 2.500000000000000000, 6.148780366869520897 ) ) ;
#26258=CONICAL_SURFACE ( 'NONE', #116126, 0.1000000000000002554, 0.003490658503988666988 ) ;
#26259=CARTESIAN_POINT ( 'NONE',  ( 1.849999999999951017, 12.50000000000000000, -6.083687093685488989 ) ) ;
#26260=CARTESIAN_POINT ( 'NONE',  ( 11.89999999999990798, 2.500000000000000000, 4.576537180435972019 ) ) ;
#26261=AXIS2_PLACEMENT_3D ( 'NONE', #9608, #412, #109072 ) ;
#26262=DIRECTION ( 'NONE',  ( 0.000000000000000000, 1.000000000000000000, 0.000000000000000000 ) ) ;
#26263=AXIS2_PLACEMENT_3D ( 'NONE', #68991, #9438, #50027 ) ;
#26264=AXIS2_PLACEMENT_3D ( 'NONE', #48012, #116090, #16581 ) ;
#26265=ORIENTED_EDGE ( 'NONE', *, *, #21941, .T. ) ;
#26266=VECTOR ( 'NONE', #68298, 1000.000000000000000 ) ;
#26267=FACE_OUTER_BOUND ( 'NONE', #90055, .T. ) ;
#26268=DIRECTION ( 'NONE',  ( 0.000000000000000000, 0.000000000000000000, 1.000000000000000000 ) ) ;
#26269=DIRECTION ( 'NONE',  ( 0.000000000000000000, 0.000000000000000000, -1.000000000000000000 ) ) ;
#26270=AXIS2_PLACEMENT_3D ( 'NONE', #42621, #51782, #82539 ) ;
#26271=DIRECTION ( 'NONE',  ( 0.000000000000000000, 0.000000000000000000, 1.000000000000000000 ) ) ;
#26272=EDGE_LOOP ( 'NONE', ( #117452, #118165 ) ) ;
#26273=ORIENTED_EDGE ( 'NONE', *, *, #19615, .T. ) ;
#26274=FACE_BOUND ( 'NONE', #21919, .T. ) ;
#26276=CARTESIAN_POINT ( 'NONE',  ( 4.399999999999937295, 12.50000000000000000, 4.048810130592458201 ) ) ;
#26277=FACE_OUTER_BOUND ( 'NONE', #23924, .T. ) ;
#26278=EDGE_LOOP ( 'NONE', ( #61470, #17760, #112952, #96892 ) ) ;
#26279=LINE ( 'NONE', #45276, #51419 ) ;
#26280=DIRECTION ( 'NONE',  ( 0.000000000000000000, -0.9999939076577903929, 0.003490651415223739937 ) ) ;
#26281=EDGE_CURVE ( 'NONE', #408, #70330, #63738, .T. ) ;
#26282=DIRECTION ( 'NONE',  ( 0.000000000000000000, 1.000000000000000000, 0.000000000000000000 ) ) ;
#26283=CARTESIAN_POINT ( 'NONE',  ( 8.349999999999923261, 12.50000000000000000, -5.802370205355749988 ) ) ;
#26284=EDGE_LOOP ( 'NONE', ( #116974, #79430, #82301, #111110 ) ) ;
#26285=CARTESIAN_POINT ( 'NONE',  ( 0.8499999999999536815, 2.500000000000000000, 5.702370205355745014 ) ) ;
#26286=EDGE_CURVE ( 'NONE', #82577, #1029, #47019, .T. ) ;
#26287=CARTESIAN_POINT ( 'NONE',  ( -7.499999999999980460, 2.500000000000000000, -4.430127018922202176 ) ) ;
#26288=FACE_OUTER_BOUND ( 'NONE', #74506, .T. ) ;
#26289=CARTESIAN_POINT ( 'NONE',  ( -11.25000000000000000, 2.500000000000000000, -7.188010851410850499 ) ) ;
#26290=CIRCLE ( 'NONE', #1142, 0.1000000000000002554 ) ;
#26291=DIRECTION ( 'NONE',  ( 0.000000000000000000, 0.000000000000000000, 1.000000000000000000 ) ) ;
#26292=ORIENTED_EDGE ( 'NONE', *, *, #30641, .T. ) ;
#26294=DIRECTION ( 'NONE',  ( 0.000000000000000000, 1.000000000000000000, 0.000000000000000000 ) ) ;
#26295=ORIENTED_EDGE ( 'NONE', *, *, #112260, .T. ) ;
#26296=DIRECTION ( 'NONE',  ( 0.000000000000000000, 0.000000000000000000, -1.000000000000000000 ) ) ;
#26297=VERTEX_POINT ( 'NONE', #72317 ) ;
#26298=ORIENTED_EDGE ( 'NONE', *, *, #86084, .T. ) ;
#26299=AXIS2_PLACEMENT_3D ( 'NONE', #90983, #664, #31432 ) ;
#26300=VERTEX_POINT ( 'NONE', #22585 ) ;
#26301=CARTESIAN_POINT ( 'NONE',  ( -10.60000000000000142, 12.50000000000000000, 0.2813168883297362810 ) ) ;
#26302=CIRCLE ( 'NONE', #103577, 0.06509327318403745899 ) ;
#26303=CIRCLE ( 'NONE', #49297, 0.1000000000000002554 ) ;
#26304=PLANE ( 'NONE',  #6614 ) ;
#26305=FACE_OUTER_BOUND ( 'NONE', #6140, .T. ) ;
#26306=CIRCLE ( 'NONE', #114310, 0.06509327318403745899 ) ;
#26309=CARTESIAN_POINT ( 'NONE',  ( 7.099999999999928590, 12.50000000000000000, 3.702399969078682407 ) ) ;
#26310=CARTESIAN_POINT ( 'NONE',  ( -11.44999999999999751, 12.50000000000000000, -2.576566944158911188 ) ) ;
#26311=EDGE_LOOP ( 'NONE', ( #30418, #1571, #79543, #122096 ) ) ;
#26312=CARTESIAN_POINT ( 'NONE',  ( -0.8000000000000381251, 2.500000000000000000, 4.330127018922196314 ) ) ;
#26313=ORIENTED_EDGE ( 'NONE', *, *, #56596, .T. ) ;
#26314=AXIS2_PLACEMENT_3D ( 'NONE', #39919, #20264, #70018 ) ;
#26315=ORIENTED_EDGE ( 'NONE', *, *, #85064, .T. ) ;
#26316=EDGE_LOOP ( 'NONE', ( #101164, #38719, #89883, #98867 ) ) ;
#26317=ORIENTED_EDGE ( 'NONE', *, *, #5782, .F. ) ;
#26318=AXIS2_PLACEMENT_3D ( 'NONE', #62836, #24843, #4522 ) ;
#26319=CONICAL_SURFACE ( 'NONE', #103677, 0.1000000000000000056, 0.003490658503988666988 ) ;
#26320=LINE ( 'NONE', #76056, #111145 ) ;
#26321=ORIENTED_EDGE ( 'NONE', *, *, #72050, .T. ) ;
#26323=ADVANCED_FACE ( 'NONE', ( #123339 ), #7412, .T. ) ;
#26324=CARTESIAN_POINT ( 'NONE',  ( 5.599999999999931255, 2.500000000000000000, 3.983716857408420076 ) ) ;
#26325=CIRCLE ( 'NONE', #28378, 0.06509327318403741736 ) ;
#26326=DIRECTION ( 'NONE',  ( 0.000000000000000000, 0.000000000000000000, 1.000000000000000000 ) ) ;
#26327=CIRCLE ( 'NONE', #109949, 0.09999999999999982514 ) ;
#26328=DIRECTION ( 'NONE',  ( 0.000000000000000000, 0.000000000000000000, 1.000000000000000000 ) ) ;
#26329=DIRECTION ( 'NONE',  ( 0.000000000000000000, 0.000000000000000000, 1.000000000000000000 ) ) ;
#26330=DIRECTION ( 'NONE',  ( 0.000000000000000000, 1.000000000000000000, 0.000000000000000000 ) ) ;
#26331=ORIENTED_EDGE ( 'NONE', *, *, #110716, .F. ) ;
#26332=DIRECTION ( 'NONE',  ( 0.000000000000000000, 1.000000000000000000, 0.000000000000000000 ) ) ;
#26333=EDGE_CURVE ( 'NONE', #100404, #2990, #15937, .T. ) ;
#26334=ORIENTED_EDGE ( 'NONE', *, *, #23375, .F. ) ;
#26335=DIRECTION ( 'NONE',  ( -0.000000000000000000, -1.000000000000000000, -0.000000000000000000 ) ) ;
#26336=ORIENTED_EDGE ( 'NONE', *, *, #40722, .F. ) ;
#26337=DIRECTION ( 'NONE',  ( 0.000000000000000000, 0.000000000000000000, -1.000000000000000000 ) ) ;
#26338=ORIENTED_EDGE ( 'NONE', *, *, #54845, .T. ) ;
#26339=EDGE_CURVE ( 'NONE', #120297, #102116, #7282, .T. ) ;
#26340=ADVANCED_FACE ( 'NONE', ( #6125 ), #25775, .T. ) ;
#26341=VERTEX_POINT ( 'NONE', #57169 ) ;
#26342=LINE ( 'NONE', #66245, #23950 ) ;
#26343=CARTESIAN_POINT ( 'NONE',  ( -11.89999999999999503, 12.50000000000000000, 3.983716857408420076 ) ) ;
#26344=CIRCLE ( 'NONE', #28401, 0.1000000000000002554 ) ;
#26345=DIRECTION ( 'NONE',  ( 0.000000000000000000, 0.000000000000000000, 1.000000000000000000 ) ) ;
#26346=AXIS2_PLACEMENT_3D ( 'NONE', #93007, #72712, #101530 ) ;
#26347=FACE_OUTER_BOUND ( 'NONE', #61603, .T. ) ;
#26348=DIRECTION ( 'NONE',  ( 0.000000000000000000, -0.9999939076577903929, 0.003490651415223739937 ) ) ;
#26349=VERTEX_POINT ( 'NONE', #74886 ) ;
#26350=LINE ( 'NONE', #63697, #70736 ) ;
#26351=PLANE ( 'NONE',  #36828 ) ;
#26353=EDGE_CURVE ( 'NONE', #33200, #68126, #13635, .T. ) ;
#26354=DIRECTION ( 'NONE',  ( 0.000000000000000000, 0.000000000000000000, -1.000000000000000000 ) ) ;
#26355=DIRECTION ( 'NONE',  ( 0.000000000000000000, -0.000000000000000000, 1.000000000000000000 ) ) ;
#26356=AXIS2_PLACEMENT_3D ( 'NONE', #94168, #23492, #33347 ) ;
#26357=CARTESIAN_POINT ( 'NONE',  ( -4.150000000000024336, 12.50000000000000000, 1.472243186433545459 ) ) ;
#26358=ORIENTED_EDGE ( 'NONE', *, *, #88826, .F. ) ;
#26359=EDGE_LOOP ( 'NONE', ( #22098, #95205, #63547, #46513 ) ) ;
#26360=VECTOR ( 'NONE', #6211, 1000.000000000000000 ) ;
#26361=CARTESIAN_POINT ( 'NONE',  ( -8.350000000000012079, 2.500000000000000000, 2.957883832488649389 ) ) ;
#26362=ORIENTED_EDGE ( 'NONE', *, *, #99245, .T. ) ;
#26363=CONICAL_SURFACE ( 'NONE', #126706, 0.09999999999999982514, 0.003490658503988666988 ) ;
#26364=DIRECTION ( 'NONE',  ( -0.000000000000000000, -1.000000000000000000, -0.000000000000000000 ) ) ;
#26365=CARTESIAN_POINT ( 'NONE',  ( -11.89999999999999680, 12.50000000000000000, -3.983716857408423628 ) ) ;
#26366=AXIS2_PLACEMENT_3D ( 'NONE', #98136, #68034, #106034 ) ;
#26367=EDGE_LOOP ( 'NONE', ( #44365, #47601 ) ) ;
#26369=CARTESIAN_POINT ( 'NONE',  ( -7.100000000000013856, 2.500000000000000000, 3.637306695894644726 ) ) ;
#26370=DIRECTION ( 'NONE',  ( -0.000000000000000000, 1.000000000000000000, -0.000000000000000000 ) ) ;
#26371=CARTESIAN_POINT ( 'NONE',  ( -7.100000000000014744, 2.500000000000000000, 4.230127018922196669 ) ) ;
#26372=CARTESIAN_POINT ( 'NONE',  ( 2.099999999999950351, 2.500000000000000000, -0.6928203230275541413 ) ) ;
#26373=VERTEX_POINT ( 'NONE', #114795 ) ;
#26374=EDGE_CURVE ( 'NONE', #51199, #12366, #1035, .T. ) ;
#26375=DIRECTION ( 'NONE',  ( -0.000000000000000000, 1.000000000000000000, -0.000000000000000000 ) ) ;
#26376=CARTESIAN_POINT ( 'NONE',  ( -4.350000000000023626, 2.500000000000000000, 1.718653347947321386 ) ) ;
#26377=EDGE_LOOP ( 'NONE', ( #81708, #19550, #106611, #116865 ) ) ;
#26378=EDGE_CURVE ( 'NONE', #71123, #1406, #34508, .T. ) ;
#26379=FACE_OUTER_BOUND ( 'NONE', #54168, .T. ) ;
#26380=CIRCLE ( 'NONE', #38929, 0.1000000000000002554 ) ;
#26381=DIRECTION ( 'NONE',  ( 0.000000000000000000, 0.000000000000000000, 1.000000000000000000 ) ) ;
#26382=ADVANCED_FACE ( 'NONE', ( #25129 ), #65036, .T. ) ;
#26383=CARTESIAN_POINT ( 'NONE',  ( 6.249999999999930722, 2.500000000000000000, 1.472243186433545459 ) ) ;
#26384=ORIENTED_EDGE ( 'NONE', *, *, #15756, .T. ) ;
#26385=AXIS2_PLACEMENT_3D ( 'NONE', #74621, #94908, #124375 ) ;
#26386=PLANE ( 'NONE',  #23933 ) ;
#26387=EDGE_CURVE ( 'NONE', #17860, #77344, #124380, .T. ) ;
#26388=EDGE_CURVE ( 'NONE', #36126, #92622, #126621, .T. ) ;
#26389=ORIENTED_EDGE ( 'NONE', *, *, #10116, .F. ) ;
#26390=FACE_OUTER_BOUND ( 'NONE', #125557, .T. ) ;
#26391=PLANE ( 'NONE',  #55063 ) ;
#26392=ADVANCED_FACE ( 'NONE', ( #75511 ), #80560, .T. ) ;
#26393=AXIS2_PLACEMENT_3D ( 'NONE', #55231, #107548, #37528 ) ;
#26394=ADVANCED_FACE ( 'NONE', ( #66970 ), #40869, .T. ) ;
#26395=CARTESIAN_POINT ( 'NONE',  ( 4.999999999999973355, 2.500000000000000000, -4.430127018922202176 ) ) ;
#26396=CIRCLE ( 'NONE', #15902, 0.09999999999999982514 ) ;
#26397=ORIENTED_EDGE ( 'NONE', *, *, #40731, .F. ) ;
#26398=CARTESIAN_POINT ( 'NONE',  ( 1.449999999999952216, 2.500000000000000000, -2.511473670974877948 ) ) ;
#26399=CIRCLE ( 'NONE', #7501, 0.06509327318403745899 ) ;
#26400=ADVANCED_FACE ( 'NONE', ( #87899 ), #36900, .T. ) ;
#26401=DIRECTION ( 'NONE',  ( -0.000000000000000000, 1.000000000000000000, -0.000000000000000000 ) ) ;
#26402=ORIENTED_EDGE ( 'NONE', *, *, #81135, .F. ) ;
#26403=VERTEX_POINT ( 'NONE', #17213 ) ;
#26404=EDGE_CURVE ( 'NONE', #79731, #48343, #116136, .T. ) ;
#26405=DIRECTION ( 'NONE',  ( -0.000000000000000000, 1.000000000000000000, -0.000000000000000000 ) ) ;
#26406=VECTOR ( 'NONE', #125544, 1000.000000000000000 ) ;
#26407=CIRCLE ( 'NONE', #112173, 0.1000000000000000472 ) ;
#26408=ORIENTED_EDGE ( 'NONE', *, *, #37320, .F. ) ;
#26409=PLANE ( 'NONE',  #50511 ) ;
#26410=CARTESIAN_POINT ( 'NONE',  ( -6.450000000000017941, 2.500000000000000000, -2.611473670974877592 ) ) ;
#26411=ORIENTED_EDGE ( 'NONE', *, *, #97949, .F. ) ;
#26412=DIRECTION ( 'NONE',  ( 0.000000000000000000, 0.000000000000000000, 1.000000000000000000 ) ) ;
#26413=CARTESIAN_POINT ( 'NONE',  ( -5.850000000000018296, 2.500000000000000000, 1.472243186433545459 ) ) ;
#26414=EDGE_LOOP ( 'NONE', ( #41732, #84710 ) ) ;
#26415=DIRECTION ( 'NONE',  ( -4.274815082592931898E-19, -0.9999939076577903929, -0.003490651415223739937 ) ) ;
#26416=CARTESIAN_POINT ( 'NONE',  ( -6.650000000000014566, 12.50000000000000000, 6.430097255199259010 ) ) ;
#26417=CARTESIAN_POINT ( 'NONE',  ( 6.449999999999931788, 12.50000000000000000, -2.446380397790840266 ) ) ;
#26418=CARTESIAN_POINT ( 'NONE',  ( -10.20000000000000284, 12.50000000000000000, -0.3464101615137782364 ) ) ;
#26419=FACE_OUTER_BOUND ( 'NONE', #8504, .T. ) ;
#26420=DIRECTION ( 'NONE',  ( 0.000000000000000000, 0.000000000000000000, 1.000000000000000000 ) ) ;
#26421=EDGE_LOOP ( 'NONE', ( #67660, #73413, #98808, #117231 ) ) ;
#26422=VERTEX_POINT ( 'NONE', #126566 ) ;
#26423=ORIENTED_EDGE ( 'NONE', *, *, #65849, .F. ) ;
#26424=EDGE_LOOP ( 'NONE', ( #17000, #20360 ) ) ;
#26425=DIRECTION ( 'NONE',  ( -0.000000000000000000, -1.000000000000000000, -0.000000000000000000 ) ) ;
#26427=DIRECTION ( 'NONE',  ( -0.000000000000000000, 1.000000000000000000, -0.000000000000000000 ) ) ;
#26428=ORIENTED_EDGE ( 'NONE', *, *, #78090, .T. ) ;
#26429=FACE_BOUND ( 'NONE', #43201, .T. ) ;
#26430=LINE ( 'NONE', #15288, #12376 ) ;
#26431=DIRECTION ( 'NONE',  ( 0.000000000000000000, 1.000000000000000000, 0.000000000000000000 ) ) ;
#26432=DIRECTION ( 'NONE',  ( -0.000000000000000000, -1.000000000000000000, -0.000000000000000000 ) ) ;
#26433=CIRCLE ( 'NONE', #124629, 0.1000000000000000056 ) ;
#26434=EDGE_CURVE ( 'NONE', #30880, #108562, #59735, .T. ) ;
#26435=DIRECTION ( 'NONE',  ( 0.000000000000000000, 0.000000000000000000, 1.000000000000000000 ) ) ;
#26436=AXIS2_PLACEMENT_3D ( 'NONE', #69314, #126326, #117120 ) ;
#26437=DIRECTION ( 'NONE',  ( 0.000000000000000000, 0.000000000000000000, 1.000000000000000000 ) ) ;
#26438=DIRECTION ( 'NONE',  ( 0.000000000000000000, -0.9999939076577903929, 0.003490651415223739937 ) ) ;
#26439=DIRECTION ( 'NONE',  ( 0.000000000000000000, 0.000000000000000000, -1.000000000000000000 ) ) ;
#26440=DIRECTION ( 'NONE',  ( -0.000000000000000000, -1.000000000000000000, -0.000000000000000000 ) ) ;
#26441=CARTESIAN_POINT ( 'NONE',  ( 13.74999999999993072, 12.50000000000000000, -2.230156782645139391 ) ) ;
#26442=DIRECTION ( 'NONE',  ( -0.000000000000000000, -1.000000000000000000, -0.000000000000000000 ) ) ;
#26443=AXIS2_PLACEMENT_3D ( 'NONE', #32184, #30249, #81880 ) ;
#26444=CONICAL_SURFACE ( 'NONE', #120435, 0.09999999999999999167, 0.003490658503988666988 ) ;
#26445=EDGE_CURVE ( 'NONE', #36155, #114467, #55511, .T. ) ;
#26446=ORIENTED_EDGE ( 'NONE', *, *, #42037, .F. ) ;
#26447=ORIENTED_EDGE ( 'NONE', *, *, #53888, .T. ) ;
#26448=ORIENTED_EDGE ( 'NONE', *, *, #89382, .F. ) ;
#26449=VERTEX_POINT ( 'NONE', #97736 ) ;
#26450=DIRECTION ( 'NONE',  ( -0.000000000000000000, 1.000000000000000000, -0.000000000000000000 ) ) ;
#26451=ORIENTED_EDGE ( 'NONE', *, *, #93004, .T. ) ;
#26452=PLANE ( 'NONE',  #123800 ) ;
#26453=ORIENTED_EDGE ( 'NONE', *, *, #98320, .T. ) ;
#26454=VERTEX_POINT ( 'NONE', #34982 ) ;
#26455=CARTESIAN_POINT ( 'NONE',  ( -6.650000000000018119, 2.500000000000000000, -2.857883832488653741 ) ) ;
#26456=VECTOR ( 'NONE', #34080, 1000.000000000000000 ) ;
#26457=AXIS2_PLACEMENT_3D ( 'NONE', #110100, #91106, #12532 ) ;
#26458=AXIS2_PLACEMENT_3D ( 'NONE', #89725, #30180, #70095 ) ;
#26459=DIRECTION ( 'NONE',  ( -4.274815082592931898E-19, -0.9999939076577903929, -0.003490651415223739937 ) ) ;
#26460=DIRECTION ( 'NONE',  ( 0.000000000000000000, -0.000000000000000000, 1.000000000000000000 ) ) ;
#26461=DIRECTION ( 'NONE',  ( 0.000000000000000000, -0.9999939076577903929, 0.003490651415223739937 ) ) ;
#26462=DIRECTION ( 'NONE',  ( 0.000000000000000000, 0.000000000000000000, 1.000000000000000000 ) ) ;
#26463=EDGE_LOOP ( 'NONE', ( #37109, #61945, #87932, #62838 ) ) ;
#26464=ORIENTED_EDGE ( 'NONE', *, *, #111511, .F. ) ;
#26465=ORIENTED_EDGE ( 'NONE', *, *, #94648, .F. ) ;
#26466=ORIENTED_EDGE ( 'NONE', *, *, #69688, .F. ) ;
#26467=DIRECTION ( 'NONE',  ( 0.000000000000000000, -0.9999939076577903929, 0.003490651415223739937 ) ) ;
#26468=ORIENTED_EDGE ( 'NONE', *, *, #129082, .F. ) ;
#26469=AXIS2_PLACEMENT_3D ( 'NONE', #38535, #128852, #20157 ) ;
#26470=ORIENTED_EDGE ( 'NONE', *, *, #69634, .F. ) ;
#26471=AXIS2_PLACEMENT_3D ( 'NONE', #27083, #125280, #55256 ) ;
#26472=PLANE ( 'NONE',  #19282 ) ;
#26473=EDGE_CURVE ( 'NONE', #2289, #23967, #114000, .T. ) ;
#26474=FACE_OUTER_BOUND ( 'NONE', #29956, .T. ) ;
#26475=CARTESIAN_POINT ( 'NONE',  ( -5.600000000000020073, 2.500000000000000000, 4.776537180435972196 ) ) ;
#26476=CIRCLE ( 'NONE', #57874, 0.06509327318403745899 ) ;
#26477=DIRECTION ( 'NONE',  ( -0.000000000000000000, -1.000000000000000000, -0.000000000000000000 ) ) ;
#26478=CARTESIAN_POINT ( 'NONE',  ( -6.450000000000019718, 2.500000000000000000, -1.818653347947326138 ) ) ;
#26479=CONICAL_SURFACE ( 'NONE', #89161, 0.1000000000000002554, 0.003490658503988666988 ) ;
#26480=DIRECTION ( 'NONE',  ( -0.000000000000000000, 1.000000000000000000, -0.000000000000000000 ) ) ;
#26481=ORIENTED_EDGE ( 'NONE', *, *, #3200, .T. ) ;
#26482=DIRECTION ( 'NONE',  ( 0.000000000000000000, -0.9999939076577903929, 0.003490651415223739937 ) ) ;
#26483=AXIS2_PLACEMENT_3D ( 'NONE', #103532, #13841, #33511 ) ;
#26484=EDGE_CURVE ( 'NONE', #53810, #47637, #49315, .T. ) ;
#26485=EDGE_LOOP ( 'NONE', ( #28987, #25712 ) ) ;
#26486=VECTOR ( 'NONE', #14937, 1000.000000000000000 ) ;
#26487=FACE_OUTER_BOUND ( 'NONE', #53735, .T. ) ;
#26488=ORIENTED_EDGE ( 'NONE', *, *, #101270, .F. ) ;
#26489=FACE_OUTER_BOUND ( 'NONE', #36565, .T. ) ;
#26490=DIRECTION ( 'NONE',  ( 0.000000000000000000, 0.000000000000000000, -1.000000000000000000 ) ) ;
#26491=ORIENTED_EDGE ( 'NONE', *, *, #88953, .F. ) ;
#26492=CARTESIAN_POINT ( 'NONE',  ( 0.6499999999999561684, 12.50000000000000000, 1.818653347947321475 ) ) ;
#26493=EDGE_CURVE ( 'NONE', #96953, #40128, #24117, .T. ) ;
#26494=DIRECTION ( 'NONE',  ( 0.000000000000000000, 0.000000000000000000, 1.000000000000000000 ) ) ;
#26496=VERTEX_POINT ( 'NONE', #129167 ) ;
#26497=VECTOR ( 'NONE', #15251, 1000.000000000000000 ) ;
#26498=AXIS2_PLACEMENT_3D ( 'NONE', #57374, #125462, #65892 ) ;
#26499=AXIS2_PLACEMENT_3D ( 'NONE', #83115, #51084, #73277 ) ;
#26500=EDGE_CURVE ( 'NONE', #54255, #120320, #22072, .T. ) ;
#26501=DIRECTION ( 'NONE',  ( 0.000000000000000000, 0.000000000000000000, -1.000000000000000000 ) ) ;
#26502=ORIENTED_EDGE ( 'NONE', *, *, #40395, .T. ) ;
#26503=EDGE_LOOP ( 'NONE', ( #31760, #6279 ) ) ;
#26504=DIRECTION ( 'NONE',  ( -4.274815082592931898E-19, -0.9999939076577903929, -0.003490651415223739937 ) ) ;
#26505=CARTESIAN_POINT ( 'NONE',  ( -7.100000000000013856, 2.500000000000000000, 5.122947341949749323 ) ) ;
#26506=EDGE_CURVE ( 'NONE', #3071, #89429, #128702, .T. ) ;
#26508=DIRECTION ( 'NONE',  ( -0.000000000000000000, -1.000000000000000000, -0.000000000000000000 ) ) ;
#26509=CARTESIAN_POINT ( 'NONE',  ( -13.74999999999998934, 12.50000000000000000, 2.857883832488652853 ) ) ;
#26510=DIRECTION ( 'NONE',  ( 0.000000000000000000, -0.000000000000000000, 1.000000000000000000 ) ) ;
#26511=AXIS2_PLACEMENT_3D ( 'NONE', #86130, #63943, #85511 ) ;
#26512=ORIENTED_EDGE ( 'NONE', *, *, #58446, .T. ) ;
#26513=DIRECTION ( 'NONE',  ( -0.000000000000000000, -1.000000000000000000, -0.000000000000000000 ) ) ;
#26514=EDGE_LOOP ( 'NONE', ( #58663, #124004 ) ) ;
#26515=CARTESIAN_POINT ( 'NONE',  ( -4.400000000000025224, 12.50000000000000000, 4.741630453620009789 ) ) ;
#26516=DIRECTION ( 'NONE',  ( 0.000000000000000000, -0.000000000000000000, 1.000000000000000000 ) ) ;
#26517=CARTESIAN_POINT ( 'NONE',  ( -6.900000000000015454, 2.500000000000000000, 4.676537180435972552 ) ) ;
#26518=EDGE_LOOP ( 'NONE', ( #46587, #64317 ) ) ;
#26519=VECTOR ( 'NONE', #53014, 1000.000000000000000 ) ;
#26520=CIRCLE ( 'NONE', #62129, 0.06509327318403745899 ) ;
#26521=CARTESIAN_POINT ( 'NONE',  ( 8.549999999999922551, 2.500000000000000000, -6.148780366869526226 ) ) ;
#26522=CARTESIAN_POINT ( 'NONE',  ( 8.349999999999919709, 2.500000000000000000, -1.472243186433550122 ) ) ;
#26523=ORIENTED_EDGE ( 'NONE', *, *, #22518, .F. ) ;
#26524=AXIS2_PLACEMENT_3D ( 'NONE', #109266, #110559, #20251 ) ;
#26525=AXIS2_PLACEMENT_3D ( 'NONE', #30934, #62949, #72138 ) ;
#26526=CARTESIAN_POINT ( 'NONE',  ( 0.1999999999999576006, 12.50000000000000000, -4.611443907251940644 ) ) ;
#26527=VERTEX_POINT ( 'NONE', #70222 ) ;
#26528=VERTEX_POINT ( 'NONE', #29651 ) ;
#26529=DIRECTION ( 'NONE',  ( 0.000000000000000000, -0.000000000000000000, 1.000000000000000000 ) ) ;
#26530=EDGE_CURVE ( 'NONE', #115201, #137, #20011, .T. ) ;
#26531=EDGE_CURVE ( 'NONE', #120872, #42274, #97268, .T. ) ;
#26532=ORIENTED_EDGE ( 'NONE', *, *, #81790, .F. ) ;
#26533=DIRECTION ( 'NONE',  ( 0.000000000000000000, 0.000000000000000000, 1.000000000000000000 ) ) ;
#26534=DIRECTION ( 'NONE',  ( -4.274815082592931898E-19, -0.9999939076577903929, -0.003490651415223739937 ) ) ;
#26536=AXIS2_PLACEMENT_3D ( 'NONE', #119541, #104724, #77681 ) ;
#26537=ADVANCED_FACE ( 'NONE', ( #90484 ), #127845, .T. ) ;
#26538=DIRECTION ( 'NONE',  ( -0.000000000000000000, 1.000000000000000000, -0.000000000000000000 ) ) ;
#26539=EDGE_LOOP ( 'NONE', ( #119856, #97790, #124865, #117989 ) ) ;
#26540=AXIS2_PLACEMENT_3D ( 'NONE', #23185, #51390, #99838 ) ;
#26541=FACE_BOUND ( 'NONE', #124401, .T. ) ;
#26542=EDGE_CURVE ( 'NONE', #1788, #40995, #48649, .T. ) ;
#26543=LINE ( 'NONE', #67071, #66715 ) ;
#26544=VERTEX_POINT ( 'NONE', #40784 ) ;
#26545=DIRECTION ( 'NONE',  ( -4.274815082592931898E-19, -0.9999939076577903929, -0.003490651415223739937 ) ) ;
#26546=DIRECTION ( 'NONE',  ( 0.000000000000000000, 1.000000000000000000, 0.000000000000000000 ) ) ;
#26547=ORIENTED_EDGE ( 'NONE', *, *, #15606, .F. ) ;
#26548=EDGE_CURVE ( 'NONE', #47717, #69367, #108838, .T. ) ;
#26549=EDGE_CURVE ( 'NONE', #95831, #10375, #167, .T. ) ;
#26550=ORIENTED_EDGE ( 'NONE', *, *, #96694, .T. ) ;
#26551=ORIENTED_EDGE ( 'NONE', *, *, #27127, .T. ) ;
#26552=DIRECTION ( 'NONE',  ( 0.000000000000000000, 1.000000000000000000, 0.000000000000000000 ) ) ;
#26553=CARTESIAN_POINT ( 'NONE',  ( -8.749999999999975131, 12.50000000000000000, 2.165063509461097713 ) ) ;
#26554=CARTESIAN_POINT ( 'NONE',  ( 4.549999999999935874, 12.50000000000000000, 6.495190528383297135 ) ) ;
#26555=FACE_BOUND ( 'NONE', #14511, .T. ) ;
#26556=ORIENTED_EDGE ( 'NONE', *, *, #116498, .T. ) ;
#26557=CIRCLE ( 'NONE', #97558, 0.1000000000000002554 ) ;
#26559=VECTOR ( 'NONE', #113197, 1000.000000000000000 ) ;
#26560=DIRECTION ( 'NONE',  ( 0.000000000000000000, 1.000000000000000000, 0.000000000000000000 ) ) ;
#26561=CARTESIAN_POINT ( 'NONE',  ( -13.34999999999999076, 12.50000000000000000, 2.165063509461101265 ) ) ;
#26562=AXIS2_PLACEMENT_3D ( 'NONE', #76673, #96941, #87123 ) ;
#26563=CARTESIAN_POINT ( 'NONE',  ( -1.850000000000033840, 2.500000000000000000, 6.741600689897071952 ) ) ;
#26564=AXIS2_PLACEMENT_3D ( 'NONE', #116051, #64998, #76132 ) ;
#26565=DIRECTION ( 'NONE',  ( 0.000000000000000000, -0.000000000000000000, 1.000000000000000000 ) ) ;
#26566=DIRECTION ( 'NONE',  ( 0.000000000000000000, -0.000000000000000000, 1.000000000000000000 ) ) ;
#26567=DIRECTION ( 'NONE',  ( -0.000000000000000000, 1.000000000000000000, -0.000000000000000000 ) ) ;
#26568=CIRCLE ( 'NONE', #110094, 0.06509327318403745899 ) ;
#26569=CARTESIAN_POINT ( 'NONE',  ( 9.149999999999916866, 2.500000000000000000, 7.188010851410848723 ) ) ;
#26570=AXIS2_PLACEMENT_3D ( 'NONE', #86784, #44944, #46219 ) ;
#26571=DIRECTION ( 'NONE',  ( -0.000000000000000000, -1.000000000000000000, -0.000000000000000000 ) ) ;
#26572=CIRCLE ( 'NONE', #74596, 0.1000000000000000472 ) ;
#26573=ORIENTED_EDGE ( 'NONE', *, *, #68946, .T. ) ;
#26574=ORIENTED_EDGE ( 'NONE', *, *, #10283, .T. ) ;
#26575=ORIENTED_EDGE ( 'NONE', *, *, #31527, .T. ) ;
#26576=VERTEX_POINT ( 'NONE', #88558 ) ;
#26577=ORIENTED_EDGE ( 'NONE', *, *, #12360, .T. ) ;
#26578=DIRECTION ( 'NONE',  ( -4.274815082592931898E-19, -0.9999939076577903929, -0.003490651415223739937 ) ) ;
#26579=CARTESIAN_POINT ( 'NONE',  ( 2.049999999999950084, 2.500000000000000000, -6.395190528383301931 ) ) ;
#26580=AXIS2_PLACEMENT_3D ( 'NONE', #23544, #62834, #42571 ) ;
#26581=VERTEX_POINT ( 'NONE', #100329 ) ;
#26582=FACE_BOUND ( 'NONE', #3885, .T. ) ;
#26583=CIRCLE ( 'NONE', #101803, 0.06509327318403745899 ) ;
#26584=CARTESIAN_POINT ( 'NONE',  ( -11.89999999999999680, 12.50000000000000000, -3.983716857408423628 ) ) ;
#26585=CONICAL_SURFACE ( 'NONE', #30803, 0.1000000000000002554, 0.003490658503988666988 ) ;
#26586=DIRECTION ( 'NONE',  ( -0.000000000000000000, -1.000000000000000000, -0.000000000000000000 ) ) ;
#26587=DIRECTION ( 'NONE',  ( -0.000000000000000000, -1.000000000000000000, -0.000000000000000000 ) ) ;
#26588=DIRECTION ( 'NONE',  ( -0.000000000000000000, 1.000000000000000000, -0.000000000000000000 ) ) ;
#26589=DIRECTION ( 'NONE',  ( 0.000000000000000000, 0.000000000000000000, 1.000000000000000000 ) ) ;
#26590=EDGE_LOOP ( 'NONE', ( #68858, #41799, #119359, #2877 ) ) ;
#26591=CARTESIAN_POINT ( 'NONE',  ( 16.32360670575004491, -2.500000000000000000, 4.874197301685487815 ) ) ;
#26593=EDGE_CURVE ( 'NONE', #125242, #59372, #57578, .T. ) ;
#26594=VERTEX_POINT ( 'NONE', #49958 ) ;
#26595=EDGE_LOOP ( 'NONE', ( #68809, #24883, #49799, #34005 ) ) ;
#26596=DIRECTION ( 'NONE',  ( -0.000000000000000000, 1.000000000000000000, -0.000000000000000000 ) ) ;
#26597=DIRECTION ( 'NONE',  ( -0.000000000000000000, 1.000000000000000000, -0.000000000000000000 ) ) ;
#26598=CARTESIAN_POINT ( 'NONE',  ( 0.8499999999999553468, 2.500000000000000000, 1.472243186433545459 ) ) ;
#26599=ORIENTED_EDGE ( 'NONE', *, *, #30228, .F. ) ;
#26600=CIRCLE ( 'NONE', #7704, 0.06509327318403745899 ) ;
#26603=DIRECTION ( 'NONE',  ( -0.000000000000000000, 1.000000000000000000, -0.000000000000000000 ) ) ;
#26605=CARTESIAN_POINT ( 'NONE',  ( -12.89999999999999147, 12.50000000000000000, 3.637306695894644726 ) ) ;
#26606=DIRECTION ( 'NONE',  ( 0.000000000000000000, 0.000000000000000000, 1.000000000000000000 ) ) ;
#26607=EDGE_LOOP ( 'NONE', ( #79685, #16950, #6915, #87391 ) ) ;
#26608=CARTESIAN_POINT ( 'NONE',  ( -3.100000000000028511, 12.50000000000000000, -4.048810130592463530 ) ) ;
#26609=CONICAL_SURFACE ( 'NONE', #68366, 0.1000000000000002554, 0.003490658503988666988 ) ;
#26610=VERTEX_POINT ( 'NONE', #89849 ) ;
#26611=AXIS2_PLACEMENT_3D ( 'NONE', #93185, #92518, #42812 ) ;
#26612=ORIENTED_EDGE ( 'NONE', *, *, #2401, .T. ) ;
#26614=CARTESIAN_POINT ( 'NONE',  ( -7.300000000000018474, 2.500000000000000000, 0.2464101615137735679 ) ) ;
#26615=DIRECTION ( 'NONE',  ( -0.000000000000000000, 1.000000000000000000, -0.000000000000000000 ) ) ;
#26616=ORIENTED_EDGE ( 'NONE', *, *, #32378, .T. ) ;
#26617=AXIS2_PLACEMENT_3D ( 'NONE', #88992, #108622, #39280 ) ;
#26618=CIRCLE ( 'NONE', #68374, 0.09999999999999982514 ) ;
#26619=VERTEX_POINT ( 'NONE', #78769 ) ;
#26620=DIRECTION ( 'NONE',  ( 0.000000000000000000, 1.000000000000000000, 0.000000000000000000 ) ) ;
#26621=CIRCLE ( 'NONE', #108174, 0.06509327318403743123 ) ;
#26622=CARTESIAN_POINT ( 'NONE',  ( 8.949999999999917577, 2.500000000000000000, -2.611473670974877592 ) ) ;
#26623=FACE_OUTER_BOUND ( 'NONE', #45978, .T. ) ;
#26624=VERTEX_POINT ( 'NONE', #80694 ) ;
#26625=VERTEX_POINT ( 'NONE', #68922 ) ;
#26626=DIRECTION ( 'NONE',  ( -4.274815082592931898E-19, -0.9999939076577903929, -0.003490651415223739937 ) ) ;
#26627=AXIS2_PLACEMENT_3D ( 'NONE', #10248, #32493, #1703 ) ;
#26628=ORIENTED_EDGE ( 'NONE', *, *, #30506, .F. ) ;
#26629=DIRECTION ( 'NONE',  ( 0.000000000000000000, 0.000000000000000000, -1.000000000000000000 ) ) ;
#26630=CONICAL_SURFACE ( 'NONE', #101846, 0.1000000000000002554, 0.003490658503988666988 ) ;
#26631=EDGE_CURVE ( 'NONE', #92524, #35250, #80037, .T. ) ;
#26632=DIRECTION ( 'NONE',  ( 0.000000000000000000, 0.000000000000000000, 1.000000000000000000 ) ) ;
#26633=VERTEX_POINT ( 'NONE', #9364 ) ;
#26634=CARTESIAN_POINT ( 'NONE',  ( -5.400000000000019895, 2.500000000000000000, 4.430127018922196847 ) ) ;
#26635=CARTESIAN_POINT ( 'NONE',  ( 7.949999999999922018, 12.50000000000000000, 6.495190528383297135 ) ) ;
#26636=DIRECTION ( 'NONE',  ( 0.000000000000000000, 1.000000000000000000, 0.000000000000000000 ) ) ;
#26637=EDGE_CURVE ( 'NONE', #49409, #8476, #119964, .T. ) ;
#26638=DIRECTION ( 'NONE',  ( -0.000000000000000000, 1.000000000000000000, -0.000000000000000000 ) ) ;
#26639=EDGE_CURVE ( 'NONE', #23744, #112624, #70865, .T. ) ;
#26640=EDGE_LOOP ( 'NONE', ( #18304, #11001 ) ) ;
#26641=DIRECTION ( 'NONE',  ( -0.000000000000000000, -1.000000000000000000, -0.000000000000000000 ) ) ;
#26642=CONICAL_SURFACE ( 'NONE', #47580, 0.09999999999999982514, 0.003490658503988666988 ) ;
#26643=CARTESIAN_POINT ( 'NONE',  ( -10.85000000000000142, 12.50000000000000000, 2.099970236277060032 ) ) ;
#26644=AXIS2_PLACEMENT_3D ( 'NONE', #15318, #34355, #64431 ) ;
#26645=EDGE_CURVE ( 'NONE', #75709, #40954, #42053, .T. ) ;
#26646=EDGE_LOOP ( 'NONE', ( #66835, #22642 ) ) ;
#26647=ADVANCED_FACE ( 'NONE', ( #103555 ), #1120, .T. ) ;
#26648=EDGE_LOOP ( 'NONE', ( #75190, #111674 ) ) ;
#26649=EDGE_CURVE ( 'NONE', #24362, #75483, #63831, .T. ) ;
#26651=DIRECTION ( 'NONE',  ( 0.000000000000000000, -0.000000000000000000, 1.000000000000000000 ) ) ;
#26652=EDGE_CURVE ( 'NONE', #75419, #125967, #2104, .T. ) ;
#26653=CARTESIAN_POINT ( 'NONE',  ( 2.500000000000002220, 1.499999999999999334, 10.00000000000000178 ) ) ;
#26654=EDGE_CURVE ( 'NONE', #3051, #97481, #122547, .T. ) ;
#26655=CARTESIAN_POINT ( 'NONE',  ( -3.150000000000033218, 12.50000000000000000, -6.841600689897078702 ) ) ;
#26656=CIRCLE ( 'NONE', #49652, 0.06509327318403745899 ) ;
#26657=FACE_OUTER_BOUND ( 'NONE', #99553, .T. ) ;
#26658=FACE_OUTER_BOUND ( 'NONE', #14856, .T. ) ;
#26659=DIRECTION ( 'NONE',  ( 0.000000000000000000, -0.000000000000000000, 1.000000000000000000 ) ) ;
#26660=DIRECTION ( 'NONE',  ( 0.000000000000000000, 0.000000000000000000, -1.000000000000000000 ) ) ;
#26661=FACE_OUTER_BOUND ( 'NONE', #69533, .T. ) ;
#26662=ADVANCED_FACE ( 'NONE', ( #83270 ), #72163, .T. ) ;
#26663=AXIS2_PLACEMENT_3D ( 'NONE', #49470, #128006, #10779 ) ;
#26664=DIRECTION ( 'NONE',  ( 0.000000000000000000, 1.000000000000000000, 0.000000000000000000 ) ) ;
#26665=EDGE_LOOP ( 'NONE', ( #83174, #59887 ) ) ;
#26666=AXIS2_PLACEMENT_3D ( 'NONE', #75903, #5224, #86359 ) ;
#26667=AXIS2_PLACEMENT_3D ( 'NONE', #28143, #88320, #6519 ) ;
#26668=ORIENTED_EDGE ( 'NONE', *, *, #6268, .T. ) ;
#26669=CARTESIAN_POINT ( 'NONE',  ( 11.04999999999991012, 2.500000000000000000, -1.818653347947326138 ) ) ;
#26670=ORIENTED_EDGE ( 'NONE', *, *, #71686, .F. ) ;
#26671=DIRECTION ( 'NONE',  ( -4.274815082592931898E-19, -0.9999939076577903929, -0.003490651415223739937 ) ) ;
#26672=FACE_OUTER_BOUND ( 'NONE', #107663, .T. ) ;
#26673=CARTESIAN_POINT ( 'NONE',  ( -6.850000000000013856, 2.500000000000000000, 1.818653347947321475 ) ) ;
#26674=ORIENTED_EDGE ( 'NONE', *, *, #47124, .F. ) ;
#26675=CARTESIAN_POINT ( 'NONE',  ( 13.74999999999989342, 12.50000000000000000, -1.472243186433550122 ) ) ;
#26676=DIRECTION ( 'NONE',  ( 0.000000000000000000, 0.000000000000000000, -1.000000000000000000 ) ) ;
#26677=DIRECTION ( 'NONE',  ( 0.000000000000000000, 0.000000000000000000, 1.000000000000000000 ) ) ;
#26678=VERTEX_POINT ( 'NONE', #123811 ) ;
#26679=CARTESIAN_POINT ( 'NONE',  ( 8.749999999999921840, 2.500000000000000000, -5.702370205355749455 ) ) ;
#26680=EDGE_LOOP ( 'NONE', ( #119051, #81086 ) ) ;
#26681=VERTEX_POINT ( 'NONE', #4040 ) ;
#26682=VERTEX_POINT ( 'NONE', #112080 ) ;
#26683=ORIENTED_EDGE ( 'NONE', *, *, #88795, .F. ) ;
#26684=CARTESIAN_POINT ( 'NONE',  ( 8.349999999999919709, 12.50000000000000000, -2.857883832488653741 ) ) ;
#26685=EDGE_CURVE ( 'NONE', #48167, #77843, #122418, .T. ) ;
#26686=CIRCLE ( 'NONE', #14147, 0.06509327318403743123 ) ;
#26687=PLANE ( 'NONE',  #50980 ) ;
#26688=DIRECTION ( 'NONE',  ( 0.000000000000000000, 1.000000000000000000, 0.000000000000000000 ) ) ;
#26689=EDGE_CURVE ( 'NONE', #47998, #50950, #53792, .T. ) ;
#26690=DIRECTION ( 'NONE',  ( 0.000000000000000000, 0.000000000000000000, 1.000000000000000000 ) ) ;
#26691=ORIENTED_EDGE ( 'NONE', *, *, #119322, .F. ) ;
#26692=ADVANCED_FACE ( 'NONE', ( #33529 ), #124460, .T. ) ;
#26693=PLANE ( 'NONE',  #64890 ) ;
#26694=ORIENTED_EDGE ( 'NONE', *, *, #10991, .F. ) ;
#26695=CARTESIAN_POINT ( 'NONE',  ( 32.15727368891349158, -2.842525632570966909, -4.549395963660428421 ) ) ;
#26696=LINE ( 'NONE', #7680, #89446 ) ;
#26697=DIRECTION ( 'NONE',  ( 0.000000000000000000, -0.000000000000000000, 1.000000000000000000 ) ) ;
#26698=CARTESIAN_POINT ( 'NONE',  ( 16.53754090007008770, -0.4856821978169225673, 6.114873053042319206 ) ) ;
#26699=EDGE_CURVE ( 'NONE', #70253, #37568, #92430, .T. ) ;
#26700=ADVANCED_FACE ( 'NONE', ( #104185 ), #111954, .T. ) ;
#26702=VECTOR ( 'NONE', #92789, 1000.000000000000000 ) ;
#26703=ADVANCED_FACE ( 'NONE', ( #13212 ), #81962, .T. ) ;
#26704=AXIS2_PLACEMENT_3D ( 'NONE', #67552, #119898, #117949 ) ;
#26705=EDGE_CURVE ( 'NONE', #119406, #65807, #45059, .T. ) ;
#26706=ORIENTED_EDGE ( 'NONE', *, *, #76930, .T. ) ;
#26707=ORIENTED_EDGE ( 'NONE', *, *, #104129, .T. ) ;
#26708=DIRECTION ( 'NONE',  ( 0.000000000000000000, 0.000000000000000000, 1.000000000000000000 ) ) ;
#26709=FACE_OUTER_BOUND ( 'NONE', #49765, .T. ) ;
#26710=CARTESIAN_POINT ( 'NONE',  ( -13.34999999999999076, 2.500000000000000000, 2.065063509461101621 ) ) ;
#26711=FACE_BOUND ( 'NONE', #92932, .T. ) ;
#26712=DIRECTION ( 'NONE',  ( 0.000000000000000000, 0.000000000000000000, 1.000000000000000000 ) ) ;
#26713=DIRECTION ( 'NONE',  ( 0.000000000000000000, 0.000000000000000000, 1.000000000000000000 ) ) ;
#26714=EDGE_CURVE ( 'NONE', #87768, #104203, #121893, .T. ) ;
#26715=AXIS2_PLACEMENT_3D ( 'NONE', #111971, #72048, #101503 ) ;
#26716=DIRECTION ( 'NONE',  ( 0.000000000000000000, 0.000000000000000000, 1.000000000000000000 ) ) ;
#26717=CARTESIAN_POINT ( 'NONE',  ( -10.45000000000000107, 2.500000000000000000, 2.065063509461097624 ) ) ;
#26718=AXIS2_PLACEMENT_3D ( 'NONE', #7432, #29035, #18547 ) ;
#26720=CARTESIAN_POINT ( 'NONE',  ( 10.39999999999991331, 2.500000000000000000, -2.385244779468109755E-15 ) ) ;
#26721=CARTESIAN_POINT ( 'NONE',  ( 12.89999999999989910, 2.500000000000000000, -0.6928203230275542523 ) ) ;
#26722=AXIS2_PLACEMENT_3D ( 'NONE', #123183, #82619, #33519 ) ;
#26723=LINE ( 'NONE', #87560, #51683 ) ;
#26724=VERTEX_POINT ( 'NONE', #121252 ) ;
#26725=ORIENTED_EDGE ( 'NONE', *, *, #21037, .F. ) ;
#26726=ORIENTED_EDGE ( 'NONE', *, *, #1179, .T. ) ;
#26727=EDGE_LOOP ( 'NONE', ( #119706, #48181, #55827, #53966 ) ) ;
#26728=FACE_OUTER_BOUND ( 'NONE', #10876, .T. ) ;
#26729=EDGE_CURVE ( 'NONE', #5370, #127196, #111411, .T. ) ;
#26730=FACE_BOUND ( 'NONE', #12871, .T. ) ;
#26731=DIRECTION ( 'NONE',  ( 0.000000000000000000, 1.000000000000000000, 0.000000000000000000 ) ) ;
#26732=CARTESIAN_POINT ( 'NONE',  ( 1.249999999999952038, 12.50000000000000000, 2.857883832488649301 ) ) ;
#26733=AXIS2_PLACEMENT_3D ( 'NONE', #13159, #123142, #126853 ) ;
#26735=DIRECTION ( 'NONE',  ( -0.000000000000000000, -1.000000000000000000, -0.000000000000000000 ) ) ;
#26737=AXIS2_PLACEMENT_3D ( 'NONE', #43382, #103582, #22457 ) ;
#26738=ORIENTED_EDGE ( 'NONE', *, *, #111770, .F. ) ;
#26739=DIRECTION ( 'NONE',  ( 0.000000000000000000, 0.000000000000000000, 1.000000000000000000 ) ) ;
#26740=CIRCLE ( 'NONE', #91586, 0.06509327318403745899 ) ;
#26741=DIRECTION ( 'NONE',  ( 0.000000000000000000, 0.000000000000000000, 1.000000000000000000 ) ) ;
#26742=CIRCLE ( 'NONE', #101963, 0.06509327318403745899 ) ;
#26743=EDGE_CURVE ( 'NONE', #123664, #68434, #72053, .T. ) ;
#26744=EDGE_LOOP ( 'NONE', ( #19866, #63870 ) ) ;
#26745=CARTESIAN_POINT ( 'NONE',  ( -8.550000000000013145, 2.500000000000000000, -6.841600689897073373 ) ) ;
#26746=CARTESIAN_POINT ( 'NONE',  ( -13.94999999999998863, 12.50000000000000000, 2.576566944158914740 ) ) ;
#26747=CIRCLE ( 'NONE', #12072, 0.06509327318403745899 ) ;
#26748=CONICAL_SURFACE ( 'NONE', #70381, 0.1000000000000002554, 0.003490658503988666988 ) ;
#26749=ORIENTED_EDGE ( 'NONE', *, *, #92145, .T. ) ;
#26750=CIRCLE ( 'NONE', #93655, 0.09999999999999982514 ) ;
#26751=LINE ( 'NONE', #39178, #101277 ) ;
#26752=PLANE ( 'NONE',  #89602 ) ;
#26754=CARTESIAN_POINT ( 'NONE',  ( -11.25000000000000000, 2.500000000000000000, 2.957883832488649389 ) ) ;
#26755=EDGE_LOOP ( 'NONE', ( #120071, #39704 ) ) ;
#26756=EDGE_LOOP ( 'NONE', ( #75788, #66354 ) ) ;
#26757=CIRCLE ( 'NONE', #116633, 0.06509327318403745899 ) ;
#26758=EDGE_CURVE ( 'NONE', #12831, #2276, #97359, .T. ) ;
#26759=DIRECTION ( 'NONE',  ( -0.000000000000000000, 1.000000000000000000, -0.000000000000000000 ) ) ;
#26761=CARTESIAN_POINT ( 'NONE',  ( 13.74999999999989875, 12.50000000000000000, 1.537336459617582918 ) ) ;
#26762=CARTESIAN_POINT ( 'NONE',  ( 3.349999999999943689, 2.500000000000000000, 2.165063509461097713 ) ) ;
#26763=AXIS2_PLACEMENT_3D ( 'NONE', #117902, #70592, #86510 ) ;
#26764=AXIS2_PLACEMENT_3D ( 'NONE', #68443, #99215, #88060 ) ;
#26765=ORIENTED_EDGE ( 'NONE', *, *, #32122, .T. ) ;
#26766=PLANE ( 'NONE',  #120730 ) ;
#26767=DIRECTION ( 'NONE',  ( -4.274815082592931898E-19, -0.9999939076577903929, -0.003490651415223739937 ) ) ;
#26768=DIRECTION ( 'NONE',  ( 0.000000000000000000, 0.000000000000000000, 1.000000000000000000 ) ) ;
#26769=CARTESIAN_POINT ( 'NONE',  ( -6.650000000000018119, 2.500000000000000000, -2.265063509461101798 ) ) ;
#26770=CARTESIAN_POINT ( 'NONE',  ( -2.900000000000030109, 2.500000000000000000, 0.6928203230275494784 ) ) ;
#26771=CARTESIAN_POINT ( 'NONE',  ( 17.50000000000000000, 2.500000000000000000, -2.922290670089280340 ) ) ;
#26772=EDGE_LOOP ( 'NONE', ( #28512, #123108, #38210, #65440 ) ) ;
#26773=VERTEX_POINT ( 'NONE', #53164 ) ;
#26774=DIRECTION ( 'NONE',  ( -0.000000000000000000, -1.000000000000000000, -0.000000000000000000 ) ) ;
#26775=CARTESIAN_POINT ( 'NONE',  ( 19.52519901027821803, -0.5909487300084481642, 4.333354523369975730 ) ) ;
#26776=DIRECTION ( 'NONE',  ( 0.000000000000000000, 0.000000000000000000, -1.000000000000000000 ) ) ;
#26777=ORIENTED_EDGE ( 'NONE', *, *, #34528, .F. ) ;
#26778=ORIENTED_EDGE ( 'NONE', *, *, #117868, .F. ) ;
#26779=ORIENTED_EDGE ( 'NONE', *, *, #50906, .F. ) ;
#26780=CARTESIAN_POINT ( 'NONE',  ( -6.250000000000017764, 2.500000000000000000, 2.757883832488649656 ) ) ;
#26781=DIRECTION ( 'NONE',  ( 0.000000000000000000, 0.000000000000000000, 1.000000000000000000 ) ) ;
#26782=CARTESIAN_POINT ( 'NONE',  ( 3.949999999999938893, 12.50000000000000000, 6.148780366869520009 ) ) ;
#26783=EDGE_CURVE ( 'NONE', #75562, #76998, #26279, .T. ) ;
#26784=PRODUCT_CONTEXT ( 'NONE', #51407, 'mechanical' ) ;
#26785=DIRECTION ( 'NONE',  ( -4.274815082592931898E-19, -0.9999939076577903929, -0.003490651415223739937 ) ) ;
#26787=AXIS2_PLACEMENT_3D ( 'NONE', #70709, #61548, #20964 ) ;
#26788=DIRECTION ( 'NONE',  ( -0.000000000000000000, -1.000000000000000000, -0.000000000000000000 ) ) ;
#26789=DIRECTION ( 'NONE',  ( -0.000000000000000000, 1.000000000000000000, -0.000000000000000000 ) ) ;
#26790=DIRECTION ( 'NONE',  ( 0.000000000000000000, 1.000000000000000000, 0.000000000000000000 ) ) ;
#26791=AXIS2_PLACEMENT_3D ( 'NONE', #12247, #82946, #40456 ) ;
#26792=CARTESIAN_POINT ( 'NONE',  ( -8.300000000000009592, 2.500000000000000000, 4.230127018922196669 ) ) ;
#26793=ADVANCED_FACE ( 'NONE', ( #4666 ), #65547, .T. ) ;
#26794=VECTOR ( 'NONE', #83920, 1000.000000000000000 ) ;
#26795=ORIENTED_EDGE ( 'NONE', *, *, #89891, .F. ) ;
#26796=DIRECTION ( 'NONE',  ( -0.000000000000000000, 1.000000000000000000, -0.000000000000000000 ) ) ;
#26797=EDGE_CURVE ( 'NONE', #94293, #98576, #101287, .T. ) ;
#26798=ORIENTED_EDGE ( 'NONE', *, *, #22890, .T. ) ;
#26799=ADVANCED_FACE ( 'NONE', ( #7252 ), #106119, .T. ) ;
#26800=VERTEX_POINT ( 'NONE', #77300 ) ;
#26801=ADVANCED_FACE ( 'NONE', ( #114640 ), #76011, .T. ) ;
#26802=LINE ( 'NONE', #66710, #77638 ) ;
#26803=DIRECTION ( 'NONE',  ( 0.000000000000000000, 0.000000000000000000, 1.000000000000000000 ) ) ;
#26805=CARTESIAN_POINT ( 'NONE',  ( -13.54999999999998828, 2.500000000000000000, 1.818653347947325472 ) ) ;
#26806=AXIS2_PLACEMENT_3D ( 'NONE', #94153, #16214, #74523 ) ;
#26807=DIRECTION ( 'NONE',  ( -0.000000000000000000, 1.000000000000000000, -0.000000000000000000 ) ) ;
#26808=CONICAL_SURFACE ( 'NONE', #83250, 0.1000000000000002554, 0.003490658503988666988 ) ;
#26809=CARTESIAN_POINT ( 'NONE',  ( 3.099999999999943245, 12.50000000000000000, 3.918623584224382839 ) ) ;
#26810=CARTESIAN_POINT ( 'NONE',  ( 5.399999999999936406, 2.500000000000000000, -5.022947341949754119 ) ) ;
#26811=CARTESIAN_POINT ( 'NONE',  ( 9.199999999999915801, 12.50000000000000000, 4.330127018922196314 ) ) ;
#26812=VERTEX_POINT ( 'NONE', #115936 ) ;
#26813=DIRECTION ( 'NONE',  ( -0.000000000000000000, 1.000000000000000000, -0.000000000000000000 ) ) ;
#26814=EDGE_CURVE ( 'NONE', #7354, #15198, #65768, .T. ) ;
#26815=CARTESIAN_POINT ( 'NONE',  ( 2.949999999999946887, 12.50000000000000000, -6.560283801567339701 ) ) ;
#26816=EDGE_CURVE ( 'NONE', #103269, #27784, #15589, .T. ) ;
#26817=ORIENTED_EDGE ( 'NONE', *, *, #117795, .F. ) ;
#26818=VECTOR ( 'NONE', #9195, 1000.000000000000000 ) ;
#26819=EDGE_CURVE ( 'NONE', #44204, #80466, #96282, .T. ) ;
#26820=ORIENTED_EDGE ( 'NONE', *, *, #115442, .F. ) ;
#26821=ORIENTED_EDGE ( 'NONE', *, *, #67216, .F. ) ;
#26822=VECTOR ( 'NONE', #74158, 1000.000000000000000 ) ;
#26824=ORIENTED_EDGE ( 'NONE', *, *, #67126, .T. ) ;
#26826=DIRECTION ( 'NONE',  ( -0.000000000000000000, 1.000000000000000000, -0.000000000000000000 ) ) ;
#26827=AXIS2_PLACEMENT_3D ( 'NONE', #28754, #8438, #28102 ) ;
#26828=EDGE_LOOP ( 'NONE', ( #117604, #6142 ) ) ;
#26829=DIRECTION ( 'NONE',  ( -4.274815082592931898E-19, -0.9999939076577903929, -0.003490651415223739937 ) ) ;
#26830=CARTESIAN_POINT ( 'NONE',  ( 17.50000000000000000, 2.750000000000000000, -2.864912725862979848 ) ) ;
#26832=CARTESIAN_POINT ( 'NONE',  ( -6.650000000000019007, 12.50000000000000000, -5.867463478539787225 ) ) ;
#26833=VERTEX_POINT ( 'NONE', #6588 ) ;
#26834=CARTESIAN_POINT ( 'NONE',  ( -3.150000000000030553, 12.50000000000000000, 6.148780366869520009 ) ) ;
#26835=CIRCLE ( 'NONE', #45718, 0.06509327318403745899 ) ;
#26836=CARTESIAN_POINT ( 'NONE',  ( 3.099999999999945466, 2.500000000000000000, 0.4464101615137735513 ) ) ;
#26837=ORIENTED_EDGE ( 'NONE', *, *, #37139, .F. ) ;
#26838=CIRCLE ( 'NONE', #51980, 0.09999999999999982514 ) ;
#26839=ORIENTED_EDGE ( 'NONE', *, *, #48495, .T. ) ;
#26840=ORIENTED_EDGE ( 'NONE', *, *, #116215, .T. ) ;
#26841=CARTESIAN_POINT ( 'NONE',  ( 11.64999999999990798, 12.50000000000000000, -1.407149913249512663 ) ) ;
#26842=AXIS2_PLACEMENT_3D ( 'NONE', #100327, #10621, #50565 ) ;
#26843=DIRECTION ( 'NONE',  ( 0.000000000000000000, -0.000000000000000000, 1.000000000000000000 ) ) ;
#26844=ORIENTED_EDGE ( 'NONE', *, *, #51171, .F. ) ;
#26845=CARTESIAN_POINT ( 'NONE',  ( 4.199999999999939782, 2.500000000000000000, 0.09999999999999772959 ) ) ;
#26846=CARTESIAN_POINT ( 'NONE',  ( 11.24999999999994316, 2.500000000000000000, -6.495190528383302464 ) ) ;
#26847=AXIS2_PLACEMENT_3D ( 'NONE', #58135, #56176, #18187 ) ;
#26848=CARTESIAN_POINT ( 'NONE',  ( -10.65000000000000391, 2.500000000000000000, -6.248780366869523206 ) ) ;
#26849=CARTESIAN_POINT ( 'NONE',  ( -7.100000000000018296, 2.500000000000000000, -4.330127018922201643 ) ) ;
#26850=ADVANCED_FACE ( 'NONE', ( #46541 ), #105496, .T. ) ;
#26851=ADVANCED_FACE ( 'NONE', ( #125118 ), #36753, .T. ) ;
#26852=VERTEX_POINT ( 'NONE', #15793 ) ;
#26853=CONICAL_SURFACE ( 'NONE', #70673, 0.09999999999999999167, 0.003490658503988666988 ) ;
#26854=CONICAL_SURFACE ( 'NONE', #108320, 0.1000000000000002554, 0.003490658503988666988 ) ;
#26855=CARTESIAN_POINT ( 'NONE',  ( 10.79999999999991012, 2.500000000000000000, -4.330127018922201643 ) ) ;
#26856=ADVANCED_FACE ( 'NONE', ( #107405 ), #1216, .T. ) ;
#26857=ORIENTED_EDGE ( 'NONE', *, *, #104116, .T. ) ;
#26858=EDGE_LOOP ( 'NONE', ( #27315, #79820, #33786, #99002 ) ) ;
#26859=ORIENTED_EDGE ( 'NONE', *, *, #74417, .T. ) ;
#26860=CARTESIAN_POINT ( 'NONE',  ( -3.749999999999994671, 2.500000000000000000, -6.495190528383302464 ) ) ;
#26861=FACE_BOUND ( 'NONE', #9223, .T. ) ;
#26862=CARTESIAN_POINT ( 'NONE',  ( 2.099999999999950351, 12.50000000000000000, -5.022947341949754119 ) ) ;
#26863=DIRECTION ( 'NONE',  ( 0.000000000000000000, 1.000000000000000000, 0.000000000000000000 ) ) ;
#26864=EDGE_CURVE ( 'NONE', #23494, #100363, #26916, .T. ) ;
#26865=DIRECTION ( 'NONE',  ( 0.000000000000000000, 1.000000000000000000, 0.000000000000000000 ) ) ;
#26866=AXIS2_PLACEMENT_3D ( 'NONE', #796, #91759, #120579 ) ;
#26867=ORIENTED_EDGE ( 'NONE', *, *, #108103, .F. ) ;
#26868=LINE ( 'NONE', #9162, #56787 ) ;
#26870=DIRECTION ( 'NONE',  ( 0.000000000000000000, 0.000000000000000000, 1.000000000000000000 ) ) ;
#26871=CARTESIAN_POINT ( 'NONE',  ( 6.249999999999932498, 2.500000000000000000, -2.757883832488654097 ) ) ;
#26872=ORIENTED_EDGE ( 'NONE', *, *, #9854, .T. ) ;
#26873=DIRECTION ( 'NONE',  ( 0.000000000000000000, 1.000000000000000000, 0.000000000000000000 ) ) ;
#26874=CONICAL_SURFACE ( 'NONE', #22960, 0.1000000000000002554, 0.003490658503988666988 ) ;
#26875=AXIS2_PLACEMENT_3D ( 'NONE', #125963, #35665, #16001 ) ;
#26876=PLANE ( 'NONE',  #62057 ) ;
#26877=CIRCLE ( 'NONE', #43617, 0.1000000000000002554 ) ;
#26878=ORIENTED_EDGE ( 'NONE', *, *, #62134, .F. ) ;
#26879=CARTESIAN_POINT ( 'NONE',  ( -6.650000000000014566, 2.500000000000000000, 5.802370205355744659 ) ) ;
#26881=ADVANCED_FACE ( 'NONE', ( #57002 ), #114092, .T. ) ;
#26882=FACE_BOUND ( 'NONE', #41541, .T. ) ;
#26883=CARTESIAN_POINT ( 'NONE',  ( 3.677964504776915167, -2.500000000000000444, -9.000000000000001776 ) ) ;
#26884=CIRCLE ( 'NONE', #83333, 0.1000000000000002554 ) ;
#26885=AXIS2_PLACEMENT_3D ( 'NONE', #79286, #119195, #69438 ) ;
#26886=VECTOR ( 'NONE', #4591, 1000.000000000000000 ) ;
#26887=ORIENTED_EDGE ( 'NONE', *, *, #68618, .T. ) ;
#26888=DIRECTION ( 'NONE',  ( 0.000000000000000000, 0.000000000000000000, 1.000000000000000000 ) ) ;
#26889=AXIS2_PLACEMENT_3D ( 'NONE', #116730, #27080, #69569 ) ;
#26890=ORIENTED_EDGE ( 'NONE', *, *, #127897, .F. ) ;
#26891=VERTEX_POINT ( 'NONE', #5331 ) ;
#26892=PLANE ( 'NONE',  #25695 ) ;
#26894=VECTOR ( 'NONE', #76944, 1000.000000000000000 ) ;
#26895=ORIENTED_EDGE ( 'NONE', *, *, #121367, .T. ) ;
#26896=CARTESIAN_POINT ( 'NONE',  ( 7.499999999999925393, 2.500000000000000000, -3.637306695894650055 ) ) ;
#26897=LINE ( 'NONE', #36730, #103598 ) ;
#26898=CONICAL_SURFACE ( 'NONE', #43640, 0.09999999999999982514, 0.003490658503988666988 ) ;
#26899=ADVANCED_FACE ( 'NONE', ( #35459 ), #47207, .T. ) ;
#26900=FACE_OUTER_BOUND ( 'NONE', #96403, .T. ) ;
#26901=DIRECTION ( 'NONE',  ( 0.000000000000000000, 0.000000000000000000, 1.000000000000000000 ) ) ;
#26902=CIRCLE ( 'NONE', #95864, 0.06509327318403745899 ) ;
#26903=VERTEX_POINT ( 'NONE', #25610 ) ;
#26904=DIRECTION ( 'NONE',  ( 0.000000000000000000, 0.000000000000000000, 1.000000000000000000 ) ) ;
#26905=DIRECTION ( 'NONE',  ( 0.000000000000000000, -0.9999939076577903929, 0.003490651415223739937 ) ) ;
#26906=LINE ( 'NONE', #17711, #86818 ) ;
#26907=CIRCLE ( 'NONE', #89606, 0.06509327318403745899 ) ;
#26908=DIRECTION ( 'NONE',  ( -0.000000000000000000, 1.000000000000000000, -0.000000000000000000 ) ) ;
#26909=ORIENTED_EDGE ( 'NONE', *, *, #61117, .T. ) ;
#26910=CARTESIAN_POINT ( 'NONE',  ( -5.850000000000018296, 12.50000000000000000, 5.802370205355744659 ) ) ;
#26911=ORIENTED_EDGE ( 'NONE', *, *, #122127, .F. ) ;
#26912=EDGE_CURVE ( 'NONE', #72066, #28200, #119156, .T. ) ;
#26913=CARTESIAN_POINT ( 'NONE',  ( 16.32360670575071993, 2.500000000000000000, 4.874197301689103590 ) ) ;
#26914=LINE ( 'NONE', #25607, #24789 ) ;
#26915=EDGE_LOOP ( 'NONE', ( #87120, #18272 ) ) ;
#26916=LINE ( 'NONE', #74728, #61876 ) ;
#26917=CARTESIAN_POINT ( 'NONE',  ( 6.699999999999930012, 2.500000000000000000, -4.330127018922201643 ) ) ;
#26918=CARTESIAN_POINT ( 'NONE',  ( 10.59999999999990905, 12.50000000000000000, 4.676537180435972552 ) ) ;
#26919=DIRECTION ( 'NONE',  ( 0.000000000000000000, 0.000000000000000000, 1.000000000000000000 ) ) ;
#26921=DIRECTION ( 'NONE',  ( -0.000000000000000000, -1.000000000000000000, -0.000000000000000000 ) ) ;
#26922=LINE ( 'NONE', #106756, #2471 ) ;
#26923=EDGE_CURVE ( 'NONE', #113934, #74025, #57657, .T. ) ;
#26925=CARTESIAN_POINT ( 'NONE',  ( 1.049999999999954525, 2.500000000000000000, -2.611473670974877592 ) ) ;
#26926=AXIS2_PLACEMENT_3D ( 'NONE', #100371, #61087, #120011 ) ;
#26927=CONICAL_SURFACE ( 'NONE', #99801, 0.1000000000000000472, 0.003490658503988666988 ) ;
#26928=FACE_OUTER_BOUND ( 'NONE', #9734, .T. ) ;
#26929=CIRCLE ( 'NONE', #58338, 0.06509327318403745899 ) ;
#26930=ORIENTED_EDGE ( 'NONE', *, *, #113745, .T. ) ;
#26931=EDGE_LOOP ( 'NONE', ( #82854, #12856, #25505, #94019 ) ) ;
#26932=DIRECTION ( 'NONE',  ( -0.000000000000000000, 1.000000000000000000, -0.000000000000000000 ) ) ;
#26934=FACE_OUTER_BOUND ( 'NONE', #51590, .T. ) ;
#26935=VERTEX_POINT ( 'NONE', #80535 ) ;
#26936=ORIENTED_EDGE ( 'NONE', *, *, #13933, .T. ) ;
#26937=ORIENTED_EDGE ( 'NONE', *, *, #29397, .F. ) ;
#26938=CIRCLE ( 'NONE', #18613, 0.09999999999999982514 ) ;
#26939=CARTESIAN_POINT ( 'NONE',  ( -3.350000000000028955, 12.50000000000000000, 7.188010851410848723 ) ) ;
#26940=CARTESIAN_POINT ( 'NONE',  ( 5.399999999999934630, 12.50000000000000000, 0.6928203230275494784 ) ) ;
#26941=CARTESIAN_POINT ( 'NONE',  ( -15.39999999999997904, 12.50000000000000000, 0.06509327318403743123 ) ) ;
#26942=ADVANCED_FACE ( 'NONE', ( #9852 ), #38694, .T. ) ;
#26944=AXIS2_PLACEMENT_3D ( 'NONE', #1379, #49868, #118575 ) ;
#26945=AXIS2_PLACEMENT_3D ( 'NONE', #95457, #15587, #78411 ) ;
#26946=DIRECTION ( 'NONE',  ( 0.000000000000000000, 0.000000000000000000, -1.000000000000000000 ) ) ;
#26947=DIRECTION ( 'NONE',  ( -0.000000000000000000, -1.000000000000000000, -0.000000000000000000 ) ) ;
#26949=ORIENTED_EDGE ( 'NONE', *, *, #77663, .T. ) ;
#26950=PLANE ( 'NONE',  #31028 ) ;
#26951=VERTEX_POINT ( 'NONE', #29497 ) ;
#26952=EDGE_CURVE ( 'NONE', #115797, #60131, #78613, .T. ) ;
#26953=VECTOR ( 'NONE', #11669, 1000.000000000000000 ) ;
#26954=ORIENTED_EDGE ( 'NONE', *, *, #108410, .F. ) ;
#26955=EDGE_LOOP ( 'NONE', ( #43415, #36488 ) ) ;
#26956=EDGE_LOOP ( 'NONE', ( #8190, #17373, #76492, #37350 ) ) ;
#26957=DIRECTION ( 'NONE',  ( 0.000000000000000000, 1.000000000000000000, 0.000000000000000000 ) ) ;
#26958=ADVANCED_FACE ( 'NONE', ( #57672 ), #74375, .T. ) ;
#26959=EDGE_LOOP ( 'NONE', ( #89965, #33716 ) ) ;
#26960=ADVANCED_FACE ( 'NONE', ( #109337 ), #61594, .T. ) ;
#26961=ORIENTED_EDGE ( 'NONE', *, *, #116023, .F. ) ;
#26962=EDGE_CURVE ( 'NONE', #74901, #43052, #49074, .T. ) ;
#26963=EDGE_CURVE ( 'NONE', #56285, #39602, #99535, .T. ) ;
#26964=DIRECTION ( 'NONE',  ( 0.000000000000000000, 0.000000000000000000, -1.000000000000000000 ) ) ;
#26965=DIRECTION ( 'NONE',  ( 0.000000000000000000, -0.9999939076577903929, 0.003490651415223739937 ) ) ;
#26966=CARTESIAN_POINT ( 'NONE',  ( 5.449999999999934452, 2.500000000000000000, 2.265063509461097357 ) ) ;
#26967=CARTESIAN_POINT ( 'NONE',  ( -2.500000000000032863, 2.500000000000000000, 5.022947341949748790 ) ) ;
#26968=EDGE_CURVE ( 'NONE', #39915, #80214, #7905, .T. ) ;
#26969=DIRECTION ( 'NONE',  ( 0.000000000000000000, -0.9999939076577903929, 0.003490651415223739937 ) ) ;
#26970=CONICAL_SURFACE ( 'NONE', #10242, 0.1000000000000002554, 0.003490658503988666988 ) ;
#26971=ORIENTED_EDGE ( 'NONE', *, *, #13553, .F. ) ;
#26972=EDGE_CURVE ( 'NONE', #104158, #85752, #124564, .T. ) ;
#26973=PLANE ( 'NONE',  #93072 ) ;
#26974=ADVANCED_FACE ( 'NONE', ( #39964 ), #129011, .T. ) ;
#26975=ORIENTED_EDGE ( 'NONE', *, *, #90892, .F. ) ;
#26976=CIRCLE ( 'NONE', #110586, 0.06509327318403745899 ) ;
#26977=CARTESIAN_POINT ( 'NONE',  ( 7.099999999999926814, 12.50000000000000000, -2.276824562219559311E-15 ) ) ;
#26978=EDGE_CURVE ( 'NONE', #12736, #122222, #55324, .T. ) ;
#26979=CONICAL_SURFACE ( 'NONE', #100135, 0.1000000000000000056, 0.003490658503988666988 ) ;
#26980=ORIENTED_EDGE ( 'NONE', *, *, #118862, .T. ) ;
#26982=ORIENTED_EDGE ( 'NONE', *, *, #10836, .F. ) ;
#26983=ORIENTED_EDGE ( 'NONE', *, *, #61075, .T. ) ;
#26984=EDGE_CURVE ( 'NONE', #82307, #127462, #9340, .T. ) ;
#26985=FACE_OUTER_BOUND ( 'NONE', #49810, .T. ) ;
#26986=AXIS2_PLACEMENT_3D ( 'NONE', #1539, #59199, #108905 ) ;
#26987=FACE_OUTER_BOUND ( 'NONE', #45738, .T. ) ;
#26988=VECTOR ( 'NONE', #20198, 1000.000000000000000 ) ;
#26989=VECTOR ( 'NONE', #118877, 1000.000000000000000 ) ;
#26990=DIRECTION ( 'NONE',  ( 0.000000000000000000, 1.000000000000000000, 0.000000000000000000 ) ) ;
#26991=DIRECTION ( 'NONE',  ( 0.000000000000000000, 0.000000000000000000, 1.000000000000000000 ) ) ;
#26992=FACE_OUTER_BOUND ( 'NONE', #120973, .T. ) ;
#26993=ORIENTED_EDGE ( 'NONE', *, *, #3459, .T. ) ;
#26994=LINE ( 'NONE', #57746, #129253 ) ;
#26995=DIRECTION ( 'NONE',  ( -0.000000000000000000, -1.000000000000000000, -0.000000000000000000 ) ) ;
#26996=DIRECTION ( 'NONE',  ( -0.000000000000000000, 1.000000000000000000, -0.000000000000000000 ) ) ;
#26997=CARTESIAN_POINT ( 'NONE',  ( 13.34999999999990017, 2.500000000000000000, 2.757883832488649656 ) ) ;
#26998=AXIS2_PLACEMENT_3D ( 'NONE', #10136, #50082, #288 ) ;
#26999=DIRECTION ( 'NONE',  ( 0.000000000000000000, 0.000000000000000000, -1.000000000000000000 ) ) ;
#27000=ORIENTED_EDGE ( 'NONE', *, *, #21140, .T. ) ;
#27001=ORIENTED_EDGE ( 'NONE', *, *, #18056, .F. ) ;
#27002=DIRECTION ( 'NONE',  ( 0.000000000000000000, 0.000000000000000000, -1.000000000000000000 ) ) ;
#27003=ORIENTED_EDGE ( 'NONE', *, *, #80200, .T. ) ;
#27004=DIRECTION ( 'NONE',  ( 0.000000000000000000, 0.000000000000000000, 1.000000000000000000 ) ) ;
#27005=DIRECTION ( 'NONE',  ( 0.000000000000000000, 0.000000000000000000, -1.000000000000000000 ) ) ;
#27006=CONICAL_SURFACE ( 'NONE', #62235, 0.1000000000000000472, 0.003490658503988666988 ) ;
#27007=AXIS2_PLACEMENT_3D ( 'NONE', #26455, #35631, #76843 ) ;
#27008=ORIENTED_EDGE ( 'NONE', *, *, #34812, .T. ) ;
#27010=CARTESIAN_POINT ( 'NONE',  ( -8.550000000000013145, 12.50000000000000000, -6.841600689897073373 ) ) ;
#27011=CARTESIAN_POINT ( 'NONE',  ( 6.449999999999933564, 2.500000000000000000, -6.741600689897078169 ) ) ;
#27013=FACE_OUTER_BOUND ( 'NONE', #47181, .T. ) ;
#27014=ORIENTED_EDGE ( 'NONE', *, *, #57837, .F. ) ;
#27015=ADVANCED_FACE ( 'NONE', ( #108044 ), #68102, .T. ) ;
#27016=DIRECTION ( 'NONE',  ( 0.000000000000000000, 0.000000000000000000, 1.000000000000000000 ) ) ;
#27017=CARTESIAN_POINT ( 'NONE',  ( -11.24999999999996447, 2.500000000000000000, -2.165063509461097713 ) ) ;
#27018=ADVANCED_FACE ( 'NONE', ( #117853 ), #28205, .T. ) ;
#27019=ORIENTED_EDGE ( 'NONE', *, *, #122862, .T. ) ;
#27020=DIRECTION ( 'NONE',  ( 0.000000000000000000, 1.000000000000000000, 0.000000000000000000 ) ) ;
#27021=CIRCLE ( 'NONE', #56254, 0.06509327318403745899 ) ;
#27022=LINE ( 'NONE', #28307, #110295 ) ;
#27023=DIRECTION ( 'NONE',  ( -0.000000000000000000, 1.000000000000000000, -0.000000000000000000 ) ) ;
#27024=VERTEX_POINT ( 'NONE', #17718 ) ;
#27025=DIRECTION ( 'NONE',  ( 0.000000000000000000, -0.000000000000000000, 1.000000000000000000 ) ) ;
#27026=ORIENTED_EDGE ( 'NONE', *, *, #46038, .T. ) ;
#27027=CARTESIAN_POINT ( 'NONE',  ( -11.24999999999996447, 2.500000000000000000, -2.165063509461097713 ) ) ;
#27028=CIRCLE ( 'NONE', #33398, 0.09999999999999982514 ) ;
#27029=CARTESIAN_POINT ( 'NONE',  ( -11.84999999999999609, 12.50000000000000000, 6.083687093685483660 ) ) ;
#27030=DIRECTION ( 'NONE',  ( 0.000000000000000000, -0.000000000000000000, 1.000000000000000000 ) ) ;
#27031=ORIENTED_EDGE ( 'NONE', *, *, #94496, .T. ) ;
#27032=CARTESIAN_POINT ( 'NONE',  ( -4.076600168545496672E-14, 12.50000000000000000, -4.957854068765716882 ) ) ;
#27033=AXIS2_PLACEMENT_3D ( 'NONE', #22022, #61290, #62584 ) ;
#27034=CARTESIAN_POINT ( 'NONE',  ( 4.149999999999939959, 2.500000000000000000, 1.372243186433545370 ) ) ;
#27035=AXIS2_PLACEMENT_3D ( 'NONE', #120758, #120119, #91296 ) ;
#27036=ORIENTED_EDGE ( 'NONE', *, *, #64476, .T. ) ;
#27037=FACE_OUTER_BOUND ( 'NONE', #126088, .T. ) ;
#27038=ORIENTED_EDGE ( 'NONE', *, *, #30386, .F. ) ;
#27039=CARTESIAN_POINT ( 'NONE',  ( -6.650000000000014566, 12.50000000000000000, 5.802370205355744659 ) ) ;
#27040=CIRCLE ( 'NONE', #102357, 0.1000000000000002554 ) ;
#27041=CIRCLE ( 'NONE', #41647, 0.06509327318403741736 ) ;
#27042=ORIENTED_EDGE ( 'NONE', *, *, #24356, .T. ) ;
#27043=DIRECTION ( 'NONE',  ( 0.000000000000000000, 1.000000000000000000, 0.000000000000000000 ) ) ;
#27044=DIRECTION ( 'NONE',  ( 0.000000000000000000, 0.000000000000000000, 1.000000000000000000 ) ) ;
#27045=ORIENTED_EDGE ( 'NONE', *, *, #95567, .T. ) ;
#27046=ORIENTED_EDGE ( 'NONE', *, *, #90165, .T. ) ;
#27047=DIRECTION ( 'NONE',  ( 0.000000000000000000, 0.000000000000000000, 1.000000000000000000 ) ) ;
#27048=CARTESIAN_POINT ( 'NONE',  ( 0.8499999999999545697, 12.50000000000000000, -1.537336459617587581 ) ) ;
#27050=CARTESIAN_POINT ( 'NONE',  ( -2.900000000000029221, 2.500000000000000000, -4.330127018922201643 ) ) ;
#27051=EDGE_CURVE ( 'NONE', #106061, #20100, #82522, .T. ) ;
#27052=CARTESIAN_POINT ( 'NONE',  ( 5.649999999999934630, 2.500000000000000000, 6.248780366869521430 ) ) ;
#27053=CARTESIAN_POINT ( 'NONE',  ( 2.299999999999948752, 2.500000000000000000, 0.4464101615137735513 ) ) ;
#27054=CONICAL_SURFACE ( 'NONE', #81439, 0.1000000000000000472, 0.003490658503988666988 ) ;
#27055=FACE_OUTER_BOUND ( 'NONE', #93708, .T. ) ;
#27056=DIRECTION ( 'NONE',  ( 0.000000000000000000, 0.000000000000000000, -1.000000000000000000 ) ) ;
#27057=DIRECTION ( 'NONE',  ( 0.000000000000000000, 1.000000000000000000, 0.000000000000000000 ) ) ;
#27058=AXIS2_PLACEMENT_3D ( 'NONE', #85593, #16819, #5727 ) ;
#27059=AXIS2_PLACEMENT_3D ( 'NONE', #96041, #27290, #117586 ) ;
#27060=EDGE_LOOP ( 'NONE', ( #41004, #31663 ) ) ;
#27062=ORIENTED_EDGE ( 'NONE', *, *, #79299, .T. ) ;
#27063=ORIENTED_EDGE ( 'NONE', *, *, #74779, .T. ) ;
#27064=DIRECTION ( 'NONE',  ( 0.000000000000000000, -0.000000000000000000, 1.000000000000000000 ) ) ;
#27065=DIRECTION ( 'NONE',  ( -0.000000000000000000, 1.000000000000000000, -0.000000000000000000 ) ) ;
#27066=ADVANCED_FACE ( 'NONE', ( #98868 ), #9203, .T. ) ;
#27067=CARTESIAN_POINT ( 'NONE',  ( -5.000000000000023093, 2.500000000000000000, 0.6928203230275494784 ) ) ;
#27068=EDGE_LOOP ( 'NONE', ( #102907, #120811, #63877, #109014 ) ) ;
#27069=FACE_BOUND ( 'NONE', #109814, .T. ) ;
#27070=EDGE_CURVE ( 'NONE', #74183, #48277, #20958, .T. ) ;
#27071=CARTESIAN_POINT ( 'NONE',  ( 9.399999999999918643, 2.500000000000000000, -0.2464101615137782308 ) ) ;
#27072=DIRECTION ( 'NONE',  ( -4.274815082592931898E-19, -0.9999939076577903929, -0.003490651415223739937 ) ) ;
#27073=AXIS2_PLACEMENT_3D ( 'NONE', #55168, #57752, #45356 ) ;
#27074=CIRCLE ( 'NONE', #1924, 0.09999999999999982514 ) ;
#27075=DIRECTION ( 'NONE',  ( -0.000000000000000000, 1.000000000000000000, -0.000000000000000000 ) ) ;
#27076=CONICAL_SURFACE ( 'NONE', #60458, 0.1000000000000002554, 0.003490658503988666988 ) ;
#27077=CARTESIAN_POINT ( 'NONE',  ( 8.549999999999922551, 2.500000000000000000, 2.511473670974873507 ) ) ;
#27078=CARTESIAN_POINT ( 'NONE',  ( -1.700000000000035261, 12.50000000000000000, 4.330127018922196314 ) ) ;
#27079=DIRECTION ( 'NONE',  ( 0.000000000000000000, 0.000000000000000000, 1.000000000000000000 ) ) ;
#27080=DIRECTION ( 'NONE',  ( -0.000000000000000000, -1.000000000000000000, -0.000000000000000000 ) ) ;
#27081=CARTESIAN_POINT ( 'NONE',  ( 6.649999999999928413, 12.50000000000000000, 1.472243186433545459 ) ) ;
#27082=EDGE_CURVE ( 'NONE', #78758, #35838, #101571, .T. ) ;
#27083=CARTESIAN_POINT ( 'NONE',  ( -1.650000000000034772, 2.500000000000000000, 5.802370205355744659 ) ) ;
#27084=CONICAL_SURFACE ( 'NONE', #20907, 0.09999999999999982514, 0.003490658503988666988 ) ;
#27085=CARTESIAN_POINT ( 'NONE',  ( 14.34999999999989306, 12.50000000000000000, -1.818653347947326138 ) ) ;
#27087=EDGE_LOOP ( 'NONE', ( #64865, #113798 ) ) ;
#27088=ORIENTED_EDGE ( 'NONE', *, *, #92381, .T. ) ;
#27089=AXIS2_PLACEMENT_3D ( 'NONE', #104296, #74194, #94459 ) ;
#27090=ORIENTED_EDGE ( 'NONE', *, *, #116959, .T. ) ;
#27091=VERTEX_POINT ( 'NONE', #81798 ) ;
#27092=CARTESIAN_POINT ( 'NONE',  ( 17.17276927100552442, -1.352216491744406834, -5.266219974095527334 ) ) ;
#27093=DIRECTION ( 'NONE',  ( 0.000000000000000000, 0.000000000000000000, 1.000000000000000000 ) ) ;
#27094=ORIENTED_EDGE ( 'NONE', *, *, #49852, .T. ) ;
#27095=VERTEX_POINT ( 'NONE', #51083 ) ;
#27096=ORIENTED_EDGE ( 'NONE', *, *, #73653, .F. ) ;
#27097=DIRECTION ( 'NONE',  ( -0.000000000000000000, -1.000000000000000000, -0.000000000000000000 ) ) ;
#27098=CARTESIAN_POINT ( 'NONE',  ( 2.500000000000002220, -2.500000000000000444, 9.000000000000001776 ) ) ;
#27099=LINE ( 'NONE', #78141, #1971 ) ;
#27100=CARTESIAN_POINT ( 'NONE',  ( -8.750000000000008882, 2.500000000000000000, 1.372243186433545370 ) ) ;
#27101=VECTOR ( 'NONE', #99709, 1000.000000000000000 ) ;
#27103=ORIENTED_EDGE ( 'NONE', *, *, #37918, .F. ) ;
#27104=ORIENTED_EDGE ( 'NONE', *, *, #67709, .T. ) ;
#27105=EDGE_CURVE ( 'NONE', #42322, #38829, #45149, .T. ) ;
#27106=VERTEX_POINT ( 'NONE', #100788 ) ;
#27107=EDGE_LOOP ( 'NONE', ( #20685, #93283 ) ) ;
#27108=FACE_OUTER_BOUND ( 'NONE', #63317, .T. ) ;
#27109=ORIENTED_EDGE ( 'NONE', *, *, #3610, .F. ) ;
#27110=EDGE_CURVE ( 'NONE', #16232, #47037, #53005, .T. ) ;
#27111=EDGE_LOOP ( 'NONE', ( #26887, #29128 ) ) ;
#27112=EDGE_CURVE ( 'NONE', #34236, #12327, #32089, .T. ) ;
#27113=CARTESIAN_POINT ( 'NONE',  ( 1.649999999999949729, 12.50000000000000000, 5.867463478539781896 ) ) ;
#27114=LINE ( 'NONE', #85387, #14038 ) ;
#27115=DIRECTION ( 'NONE',  ( 0.000000000000000000, 0.000000000000000000, 1.000000000000000000 ) ) ;
#27116=DIRECTION ( 'NONE',  ( -0.000000000000000000, -1.000000000000000000, -0.000000000000000000 ) ) ;
#27117=EDGE_CURVE ( 'NONE', #26581, #125089, #51216, .T. ) ;
#27118=ADVANCED_FACE ( 'NONE', ( #72005 ), #40762, .T. ) ;
#27120=AXIS2_PLACEMENT_3D ( 'NONE', #85041, #86325, #36619 ) ;
#27121=ADVANCED_FACE ( 'NONE', ( #83747 ), #21608, .T. ) ;
#27122=EDGE_LOOP ( 'NONE', ( #80049, #65049, #77633, #99071 ) ) ;
#27123=DIRECTION ( 'NONE',  ( 0.000000000000000000, 0.000000000000000000, -1.000000000000000000 ) ) ;
#27124=EDGE_LOOP ( 'NONE', ( #66394, #100874 ) ) ;
#27125=DIRECTION ( 'NONE',  ( -0.000000000000000000, -1.000000000000000000, -0.000000000000000000 ) ) ;
#27126=AXIS2_PLACEMENT_3D ( 'NONE', #73664, #44881, #113604 ) ;
#27127=EDGE_CURVE ( 'NONE', #29239, #55712, #99329, .T. ) ;
#27128=ORIENTED_EDGE ( 'NONE', *, *, #117518, .T. ) ;
#27129=CARTESIAN_POINT ( 'NONE',  ( 14.39999999999989555, 12.50000000000000000, -0.4115034346978156399 ) ) ;
#27130=CARTESIAN_POINT ( 'NONE',  ( 7.299999999999927880, 2.500000000000000000, 3.983716857408420964 ) ) ;
#27131=EDGE_LOOP ( 'NONE', ( #23207, #86488, #17903, #29356 ) ) ;
#27132=AXIS2_PLACEMENT_3D ( 'NONE', #40783, #18532, #81332 ) ;
#27133=CARTESIAN_POINT ( 'NONE',  ( -0.4500000000000402012, 12.50000000000000000, 6.430097255199259010 ) ) ;
#27134=CARTESIAN_POINT ( 'NONE',  ( -1.700000000000034817, 2.500000000000000000, -2.385244779468109755E-15 ) ) ;
#27135=ORIENTED_EDGE ( 'NONE', *, *, #15225, .F. ) ;
#27136=ADVANCED_FACE ( 'NONE', ( #121727 ), #61679, .T. ) ;
#27137=AXIS2_PLACEMENT_3D ( 'NONE', #71084, #110986, #111661 ) ;
#27138=AXIS2_PLACEMENT_3D ( 'NONE', #25553, #93032, #85129 ) ;
#27139=DIRECTION ( 'NONE',  ( 0.000000000000000000, 1.000000000000000000, 0.000000000000000000 ) ) ;
#27140=ORIENTED_EDGE ( 'NONE', *, *, #303, .T. ) ;
#27141=ORIENTED_EDGE ( 'NONE', *, *, #108780, .T. ) ;
#27142=DIRECTION ( 'NONE',  ( 0.000000000000000000, 0.000000000000000000, -1.000000000000000000 ) ) ;
#27143=CARTESIAN_POINT ( 'NONE',  ( -4.119968255444916849E-14, 2.500000000000000000, 3.637306695894644726 ) ) ;
#27145=CARTESIAN_POINT ( 'NONE',  ( -10.40000000000000391, 2.500000000000000000, -3.637306695894645614 ) ) ;
#27146=PLANE ( 'NONE',  #62502 ) ;
#27147=DIRECTION ( 'NONE',  ( -0.000000000000000000, 1.000000000000000000, -0.000000000000000000 ) ) ;
#27148=ORIENTED_EDGE ( 'NONE', *, *, #116079, .F. ) ;
#27149=FACE_OUTER_BOUND ( 'NONE', #82157, .T. ) ;
#27150=CIRCLE ( 'NONE', #33430, 0.06509327318403745899 ) ;
#27151=ORIENTED_EDGE ( 'NONE', *, *, #21058, .F. ) ;
#27152=DIRECTION ( 'NONE',  ( 0.000000000000000000, 0.000000000000000000, 1.000000000000000000 ) ) ;
#27153=DIRECTION ( 'NONE',  ( 0.000000000000000000, 1.000000000000000000, 0.000000000000000000 ) ) ;
#27154=CARTESIAN_POINT ( 'NONE',  ( 1.899999999999951283, 2.500000000000000000, -3.983716857408426293 ) ) ;
#27155=FACE_OUTER_BOUND ( 'NONE', #115714, .T. ) ;
#27156=CARTESIAN_POINT ( 'NONE',  ( 3.949999999999941558, 2.500000000000000000, -6.248780366869526759 ) ) ;
#27157=EDGE_LOOP ( 'NONE', ( #33847, #119219 ) ) ;
#27158=AXIS2_PLACEMENT_3D ( 'NONE', #51905, #122574, #64283 ) ;
#27159=ADVANCED_FACE ( 'NONE', ( #81173 ), #3889, .T. ) ;
#27160=CARTESIAN_POINT ( 'NONE',  ( 10.84999999999990905, 12.50000000000000000, 2.165063509461097713 ) ) ;
#27161=FACE_OUTER_BOUND ( 'NONE', #64288, .T. ) ;
#27162=CIRCLE ( 'NONE', #104528, 0.09999999999999999167 ) ;
#27163=ORIENTED_EDGE ( 'NONE', *, *, #42509, .F. ) ;
#27164=CARTESIAN_POINT ( 'NONE',  ( 8.349999999999919709, 2.500000000000000000, 7.188010851410848723 ) ) ;
#27165=ADVANCED_FACE ( 'NONE', ( #43847 ), #115951, .T. ) ;
#27166=CIRCLE ( 'NONE', #43911, 0.06509327318403745899 ) ;
#27167=CIRCLE ( 'NONE', #108733, 0.1000000000000002554 ) ;
#27168=ORIENTED_EDGE ( 'NONE', *, *, #122381, .F. ) ;
#27169=ORIENTED_EDGE ( 'NONE', *, *, #78851, .T. ) ;
#27170=CARTESIAN_POINT ( 'NONE',  ( -4.293440603042597559E-14, 12.50000000000000000, 5.022947341949748790 ) ) ;
#27171=ORIENTED_EDGE ( 'NONE', *, *, #14565, .T. ) ;
#27172=DIRECTION ( 'NONE',  ( -0.000000000000000000, -1.000000000000000000, -0.000000000000000000 ) ) ;
#27173=DIRECTION ( 'NONE',  ( 0.000000000000000000, -0.000000000000000000, 1.000000000000000000 ) ) ;
#27174=AXIS2_PLACEMENT_3D ( 'NONE', #77066, #84943, #75129 ) ;
#27175=PLANE ( 'NONE',  #75162 ) ;
#27176=VERTEX_POINT ( 'NONE', #123648 ) ;
#27177=FACE_BOUND ( 'NONE', #72497, .T. ) ;
#27178=CARTESIAN_POINT ( 'NONE',  ( 7.699999999999923794, 2.500000000000000000, -0.2464101615137783419 ) ) ;
#27179=EDGE_LOOP ( 'NONE', ( #116456, #119569 ) ) ;
#27180=CARTESIAN_POINT ( 'NONE',  ( -9.550000000000007816, 2.500000000000000000, -6.595190528383296780 ) ) ;
#27181=CARTESIAN_POINT ( 'NONE',  ( -8.300000000000011369, 12.50000000000000000, -4.265033745738164406 ) ) ;
#27182=ORIENTED_EDGE ( 'NONE', *, *, #103171, .F. ) ;
#27183=EDGE_LOOP ( 'NONE', ( #52562, #70624, #101635, #65915 ) ) ;
#27184=ORIENTED_EDGE ( 'NONE', *, *, #44877, .F. ) ;
#27185=CARTESIAN_POINT ( 'NONE',  ( -0.2000000000000399791, 12.50000000000000000, -4.741630453620015118 ) ) ;
#27186=DIRECTION ( 'NONE',  ( -4.274815082592931898E-19, -0.9999939076577903929, -0.003490651415223739937 ) ) ;
#27187=DIRECTION ( 'NONE',  ( 0.000000000000000000, 1.000000000000000000, 0.000000000000000000 ) ) ;
#27188=FACE_BOUND ( 'NONE', #64721, .T. ) ;
#27189=VERTEX_POINT ( 'NONE', #33378 ) ;
#27190=DIRECTION ( 'NONE',  ( 0.000000000000000000, 1.000000000000000000, 0.000000000000000000 ) ) ;
#27191=DIRECTION ( 'NONE',  ( 0.000000000000000000, 0.000000000000000000, -1.000000000000000000 ) ) ;
#27192=VERTEX_POINT ( 'NONE', #103392 ) ;
#27193=EDGE_CURVE ( 'NONE', #48991, #58714, #67921, .T. ) ;
#27194=DIRECTION ( 'NONE',  ( 0.000000000000000000, 0.000000000000000000, -1.000000000000000000 ) ) ;
#27195=CARTESIAN_POINT ( 'NONE',  ( 7.899999999999924860, 2.500000000000000000, -5.122947341949753763 ) ) ;
#27196=DIRECTION ( 'NONE',  ( 0.000000000000000000, 1.000000000000000000, 0.000000000000000000 ) ) ;
#27197=AXIS2_PLACEMENT_3D ( 'NONE', #89561, #18880, #524 ) ;
#27198=CARTESIAN_POINT ( 'NONE',  ( 14.54999999999989235, 12.50000000000000000, -2.165063509461101710 ) ) ;
#27199=DIRECTION ( 'NONE',  ( 0.000000000000000000, -0.000000000000000000, 1.000000000000000000 ) ) ;
#27200=EDGE_CURVE ( 'NONE', #93869, #91958, #101384, .T. ) ;
#27201=AXIS2_PLACEMENT_3D ( 'NONE', #127303, #37637, #77536 ) ;
#27202=AXIS2_PLACEMENT_3D ( 'NONE', #59908, #19962, #293 ) ;
#27203=ORIENTED_EDGE ( 'NONE', *, *, #32506, .F. ) ;
#27204=VERTEX_POINT ( 'NONE', #93570 ) ;
#27205=ORIENTED_EDGE ( 'NONE', *, *, #44883, .T. ) ;
#27206=ORIENTED_EDGE ( 'NONE', *, *, #69665, .T. ) ;
#27207=ORIENTED_EDGE ( 'NONE', *, *, #3242, .T. ) ;
#27208=DIRECTION ( 'NONE',  ( -4.274815082592931898E-19, -0.9999939076577903929, -0.003490651415223739937 ) ) ;
#27209=ADVANCED_FACE ( 'NONE', ( #110624 ), #128598, .T. ) ;
#27210=CARTESIAN_POINT ( 'NONE',  ( -2.500000000000032419, 12.50000000000000000, -3.637306695894650055 ) ) ;
#27211=ORIENTED_EDGE ( 'NONE', *, *, #101283, .F. ) ;
#27212=FACE_BOUND ( 'NONE', #95823, .T. ) ;
#27213=ADVANCED_FACE ( 'NONE', ( #11775 ), #32454, .T. ) ;
#27214=LINE ( 'NONE', #127366, #35276 ) ;
#27215=CONICAL_SURFACE ( 'NONE', #87751, 0.1000000000000002554, 0.003490658503988666988 ) ;
#27216=EDGE_CURVE ( 'NONE', #124539, #104801, #26166, .T. ) ;
#27217=DIRECTION ( 'NONE',  ( 0.000000000000000000, 1.000000000000000000, 0.000000000000000000 ) ) ;
#27218=CARTESIAN_POINT ( 'NONE',  ( -3.150000000000029221, 2.500000000000000000, -1.818653347947326138 ) ) ;
#27219=CARTESIAN_POINT ( 'NONE',  ( -11.64999999999999680, 2.500000000000000000, -2.165063509461097713 ) ) ;
#27220=EDGE_CURVE ( 'NONE', #100479, #71602, #95499, .T. ) ;
#27221=DIRECTION ( 'NONE',  ( 0.000000000000000000, -0.9999939076577903929, 0.003490651415223739937 ) ) ;
#27222=VERTEX_POINT ( 'NONE', #64102 ) ;
#27223=DIRECTION ( 'NONE',  ( 0.000000000000000000, 0.000000000000000000, 1.000000000000000000 ) ) ;
#27224=ORIENTED_EDGE ( 'NONE', *, *, #86047, .F. ) ;
#27225=EDGE_LOOP ( 'NONE', ( #56125, #73003, #40779, #3489 ) ) ;
#27226=VERTEX_POINT ( 'NONE', #113857 ) ;
#27227=CARTESIAN_POINT ( 'NONE',  ( -7.499999999999980460, 2.500000000000000000, -2.276824562219559311E-15 ) ) ;
#27228=CARTESIAN_POINT ( 'NONE',  ( 15.62876697814534133, 2.499999999999999112, 5.624417669420174626 ) ) ;
#27229=DIRECTION ( 'NONE',  ( 0.000000000000000000, -0.9999939076577903929, 0.003490651415223739937 ) ) ;
#27230=ORIENTED_EDGE ( 'NONE', *, *, #128621, .T. ) ;
#27231=CARTESIAN_POINT ( 'NONE',  ( 12.64862127267500114, 2.500000000000000444, -8.430718249866270497 ) ) ;
#27232=CIRCLE ( 'NONE', #81610, 0.06509327318403745899 ) ;
#27233=CARTESIAN_POINT ( 'NONE',  ( 105.5000000000000142, 2.449293598294706414E-16, -2.000000000000000000 ) ) ;
#27234=VECTOR ( 'NONE', #57178, 1000.000000000000000 ) ;
#27235=FACE_OUTER_BOUND ( 'NONE', #7983, .T. ) ;
#27237=FACE_OUTER_BOUND ( 'NONE', #55911, .T. ) ;
#27238=DIRECTION ( 'NONE',  ( 0.000000000000000000, 0.000000000000000000, 1.000000000000000000 ) ) ;
#27239=LINE ( 'NONE', #7599, #74622 ) ;
#27240=VERTEX_POINT ( 'NONE', #64743 ) ;
#27241=CARTESIAN_POINT ( 'NONE',  ( -0.8000000000000315747, 2.500000000000000000, -0.1000000000000000056 ) ) ;
#27242=AXIS2_PLACEMENT_3D ( 'NONE', #14901, #43140, #33939 ) ;
#27243=VERTEX_POINT ( 'NONE', #54918 ) ;
#27244=ADVANCED_FACE ( 'NONE', ( #35933 ), #78413, .T. ) ;
#27245=VERTEX_POINT ( 'NONE', #46383 ) ;
#27246=CARTESIAN_POINT ( 'NONE',  ( -9.200000000000009948, 2.500000000000000000, -4.230127018922197557 ) ) ;
#27247=DIRECTION ( 'NONE',  ( 0.000000000000000000, 0.000000000000000000, 1.000000000000000000 ) ) ;
#27248=FACE_OUTER_BOUND ( 'NONE', #8516, .T. ) ;
#27249=ORIENTED_EDGE ( 'NONE', *, *, #14352, .F. ) ;
#27250=ORIENTED_EDGE ( 'NONE', *, *, #94826, .F. ) ;
#27251=EDGE_CURVE ( 'NONE', #44951, #14963, #107642, .T. ) ;
#27252=DIRECTION ( 'NONE',  ( 0.000000000000000000, 0.000000000000000000, -1.000000000000000000 ) ) ;
#27253=CARTESIAN_POINT ( 'NONE',  ( -2.050000000000032685, 12.50000000000000000, -6.495190528383302464 ) ) ;
#27254=LINE ( 'NONE', #10209, #87915 ) ;
#27255=EDGE_LOOP ( 'NONE', ( #11006, #90893, #115057, #83284 ) ) ;
#27256=ORIENTED_EDGE ( 'NONE', *, *, #50270, .T. ) ;
#27257=ADVANCED_FACE ( 'NONE', ( #96769 ), #59555, .T. ) ;
#27258=DIRECTION ( 'NONE',  ( -0.000000000000000000, -1.000000000000000000, -0.000000000000000000 ) ) ;
#27259=ADVANCED_FACE ( 'NONE', ( #124962 ), #21977, .T. ) ;
#27260=CIRCLE ( 'NONE', #12593, 0.06509327318403745899 ) ;
#27261=EDGE_CURVE ( 'NONE', #1609, #74070, #106600, .T. ) ;
#27262=VERTEX_POINT ( 'NONE', #35304 ) ;
#27263=DIRECTION ( 'NONE',  ( -0.000000000000000000, 1.000000000000000000, -0.000000000000000000 ) ) ;
#27264=CARTESIAN_POINT ( 'NONE',  ( -1.650000000000034772, 12.50000000000000000, 6.430097255199259010 ) ) ;
#27265=ORIENTED_EDGE ( 'NONE', *, *, #69092, .T. ) ;
#27266=LINE ( 'NONE', #18093, #73296 ) ;
#27267=ADVANCED_FACE ( 'NONE', ( #75213 ), #3093, .T. ) ;
#27268=DIRECTION ( 'NONE',  ( 0.000000000000000000, -0.000000000000000000, 1.000000000000000000 ) ) ;
#27269=AXIS2_PLACEMENT_3D ( 'NONE', #32057, #72613, #100753 ) ;
#27270=DIRECTION ( 'NONE',  ( 0.000000000000000000, 0.000000000000000000, 1.000000000000000000 ) ) ;
#27271=DIRECTION ( 'NONE',  ( -4.274815082592931898E-19, -0.9999939076577903929, -0.003490651415223739937 ) ) ;
#27272=VERTEX_POINT ( 'NONE', #26761 ) ;
#27273=EDGE_CURVE ( 'NONE', #120531, #2500, #118094, .T. ) ;
#27274=CARTESIAN_POINT ( 'NONE',  ( 10.84999999999990905, 2.500000000000000000, -7.188010851410854052 ) ) ;
#27275=EDGE_CURVE ( 'NONE', #115252, #112245, #28222, .T. ) ;
#27276=CARTESIAN_POINT ( 'NONE',  ( 8.349999999999919709, 12.50000000000000000, 6.495190528383297135 ) ) ;
#27277=VERTEX_POINT ( 'NONE', #5169 ) ;
#27278=ORIENTED_EDGE ( 'NONE', *, *, #42244, .T. ) ;
#27280=DIRECTION ( 'NONE',  ( -0.000000000000000000, -1.000000000000000000, -0.000000000000000000 ) ) ;
#27281=DIRECTION ( 'NONE',  ( 0.000000000000000000, 1.000000000000000000, 0.000000000000000000 ) ) ;
#27282=DIRECTION ( 'NONE',  ( -4.274815082592931898E-19, -0.9999939076577903929, -0.003490651415223739937 ) ) ;
#27284=DIRECTION ( 'NONE',  ( -0.000000000000000000, -1.000000000000000000, -0.000000000000000000 ) ) ;
#27285=CARTESIAN_POINT ( 'NONE',  ( -5.450000000000023270, 12.50000000000000000, -6.495190528383302464 ) ) ;
#27286=DIRECTION ( 'NONE',  ( 0.000000000000000000, 0.000000000000000000, 1.000000000000000000 ) ) ;
#27287=DIRECTION ( 'NONE',  ( 0.000000000000000000, 0.000000000000000000, -1.000000000000000000 ) ) ;
#27288=CIRCLE ( 'NONE', #8409, 0.06509327318403745899 ) ;
#27289=AXIS2_PLACEMENT_3D ( 'NONE', #34531, #35799, #73780 ) ;
#27290=DIRECTION ( 'NONE',  ( -0.000000000000000000, 1.000000000000000000, -0.000000000000000000 ) ) ;
#27291=CIRCLE ( 'NONE', #23180, 0.06509327318403745899 ) ;
#27292=ORIENTED_EDGE ( 'NONE', *, *, #53560, .T. ) ;
#27293=CARTESIAN_POINT ( 'NONE',  ( 7.099999999999928590, 2.500000000000000000, -5.022947341949754119 ) ) ;
#27294=DIRECTION ( 'NONE',  ( -0.000000000000000000, -1.000000000000000000, -0.000000000000000000 ) ) ;
#27295=CARTESIAN_POINT ( 'NONE',  ( 9.349999999999919709, 12.50000000000000000, 2.511473670974873507 ) ) ;
#27296=DIRECTION ( 'NONE',  ( 0.000000000000000000, 1.000000000000000000, 0.000000000000000000 ) ) ;
#27297=VERTEX_POINT ( 'NONE', #115110 ) ;
#27298=DIRECTION ( 'NONE',  ( 0.000000000000000000, 1.000000000000000000, 0.000000000000000000 ) ) ;
#27299=CARTESIAN_POINT ( 'NONE',  ( 8.549999999999918998, 2.500000000000000000, -1.718653347947326049 ) ) ;
#27300=DIRECTION ( 'NONE',  ( 0.000000000000000000, 1.000000000000000000, 0.000000000000000000 ) ) ;
#27301=EDGE_LOOP ( 'NONE', ( #65119, #27505 ) ) ;
#27302=EDGE_LOOP ( 'NONE', ( #110395, #49845 ) ) ;
#27303=EDGE_CURVE ( 'NONE', #120069, #53996, #125587, .T. ) ;
#27304=ORIENTED_EDGE ( 'NONE', *, *, #6011, .F. ) ;
#27305=ORIENTED_EDGE ( 'NONE', *, *, #88739, .T. ) ;
#27306=ORIENTED_EDGE ( 'NONE', *, *, #93980, .F. ) ;
#27307=FACE_OUTER_BOUND ( 'NONE', #69277, .T. ) ;
#27308=DIRECTION ( 'NONE',  ( -0.000000000000000000, -1.000000000000000000, -0.000000000000000000 ) ) ;
#27309=DIRECTION ( 'NONE',  ( 0.000000000000000000, 0.000000000000000000, 1.000000000000000000 ) ) ;
#27310=DIRECTION ( 'NONE',  ( -0.000000000000000000, 1.000000000000000000, -0.000000000000000000 ) ) ;
#27311=AXIS2_PLACEMENT_3D ( 'NONE', #20382, #102162, #51143 ) ;
#27312=ORIENTED_EDGE ( 'NONE', *, *, #9051, .T. ) ;
#27313=AXIS2_PLACEMENT_3D ( 'NONE', #119669, #534, #52236 ) ;
#27314=DIRECTION ( 'NONE',  ( 0.000000000000000000, 0.000000000000000000, 1.000000000000000000 ) ) ;
#27315=ORIENTED_EDGE ( 'NONE', *, *, #113985, .F. ) ;
#27316=CARTESIAN_POINT ( 'NONE',  ( 48.83465639049822471, -3.619824997336297034, -4.313881469032290639 ) ) ;
#27317=CARTESIAN_POINT ( 'NONE',  ( 7.899999999999923084, 12.50000000000000000, 0.6928203230275494784 ) ) ;
#27318=CYLINDRICAL_SURFACE ( 'NONE', #12884, 1.000000000000000888 ) ;
#27319=DIRECTION ( 'NONE',  ( -0.000000000000000000, -1.000000000000000000, -0.000000000000000000 ) ) ;
#27320=FACE_OUTER_BOUND ( 'NONE', #103058, .T. ) ;
#27321=AXIS2_PLACEMENT_3D ( 'NONE', #41689, #81586, #41048 ) ;
#27322=ORIENTED_EDGE ( 'NONE', *, *, #121067, .F. ) ;
#27323=ORIENTED_EDGE ( 'NONE', *, *, #69970, .F. ) ;
#27324=ORIENTED_EDGE ( 'NONE', *, *, #34857, .F. ) ;
#27325=ORIENTED_EDGE ( 'NONE', *, *, #13362, .T. ) ;
#27326=PLANE ( 'NONE',  #39807 ) ;
#27327=CARTESIAN_POINT ( 'NONE',  ( 8.149999999999920419, 2.500000000000000000, 6.148780366869520897 ) ) ;
#27328=CARTESIAN_POINT ( 'NONE',  ( 11.44999999999990692, 12.50000000000000000, 1.818653347947321475 ) ) ;
#27329=FACE_BOUND ( 'NONE', #8427, .T. ) ;
#27330=DIRECTION ( 'NONE',  ( 0.000000000000000000, 1.000000000000000000, 0.000000000000000000 ) ) ;
#27331=DIRECTION ( 'NONE',  ( 0.000000000000000000, 0.000000000000000000, 1.000000000000000000 ) ) ;
#27332=DIRECTION ( 'NONE',  ( -0.000000000000000000, -1.000000000000000000, -0.000000000000000000 ) ) ;
#27333=FACE_OUTER_BOUND ( 'NONE', #46042, .T. ) ;
#27334=AXIS2_PLACEMENT_3D ( 'NONE', #48413, #18302, #88987 ) ;
#27335=CIRCLE ( 'NONE', #4338, 0.06509327318403745899 ) ;
#27337=DIRECTION ( 'NONE',  ( 0.000000000000000000, 0.000000000000000000, 1.000000000000000000 ) ) ;
#27338=PLANE ( 'NONE',  #76200 ) ;
#27339=VECTOR ( 'NONE', #64693, 1000.000000000000000 ) ;
#27340=EDGE_CURVE ( 'NONE', #94406, #55939, #4503, .T. ) ;
#27341=DIRECTION ( 'NONE',  ( -0.000000000000000000, -1.000000000000000000, -0.000000000000000000 ) ) ;
#27342=EDGE_LOOP ( 'NONE', ( #109241, #57851, #47838, #41683 ) ) ;
#27343=CIRCLE ( 'NONE', #108914, 0.1000000000000002554 ) ;
#27344=VERTEX_POINT ( 'NONE', #84389 ) ;
#27345=EDGE_LOOP ( 'NONE', ( #71703, #113714 ) ) ;
#27346=ORIENTED_EDGE ( 'NONE', *, *, #114143, .T. ) ;
#27347=EDGE_CURVE ( 'NONE', #59613, #42850, #122320, .T. ) ;
#27348=CARTESIAN_POINT ( 'NONE',  ( -10.00000000000000533, 12.50000000000000000, 5.022947341949748790 ) ) ;
#27349=FACE_BOUND ( 'NONE', #41552, .T. ) ;
#27350=EDGE_CURVE ( 'NONE', #58766, #33854, #65862, .T. ) ;
#27351=DIRECTION ( 'NONE',  ( 0.000000000000000000, -0.000000000000000000, 1.000000000000000000 ) ) ;
#27352=DIRECTION ( 'NONE',  ( -0.000000000000000000, 1.000000000000000000, -0.000000000000000000 ) ) ;
#27353=EDGE_CURVE ( 'NONE', #10496, #94042, #109702, .T. ) ;
#27354=ADVANCED_FACE ( 'NONE', ( #104657 ), #14968, .T. ) ;
#27355=EDGE_LOOP ( 'NONE', ( #109821, #10068, #67069, #25256 ) ) ;
#27356=CARTESIAN_POINT ( 'NONE',  ( -3.550000000000027356, 2.500000000000000000, 1.918653347947321564 ) ) ;
#27357=ADVANCED_FACE ( 'NONE', ( #10339 ), #47012, .T. ) ;
#27358=DIRECTION ( 'NONE',  ( -0.000000000000000000, -1.000000000000000000, -0.000000000000000000 ) ) ;
#27359=ADVANCED_FACE ( 'NONE', ( #18861 ), #80463, .T. ) ;
#27360=CARTESIAN_POINT ( 'NONE',  ( 0.6499999999999566125, 12.50000000000000000, -6.148780366869526226 ) ) ;
#27361=VERTEX_POINT ( 'NONE', #109834 ) ;
#27362=CARTESIAN_POINT ( 'NONE',  ( 13.34999999999989662, 12.50000000000000000, -2.857883832488653741 ) ) ;
#27363=DIRECTION ( 'NONE',  ( -4.274815082592931898E-19, -0.9999939076577903929, -0.003490651415223739937 ) ) ;
#27364=AXIS2_PLACEMENT_3D ( 'NONE', #74292, #114210, #4876 ) ;
#27365=ORIENTED_EDGE ( 'NONE', *, *, #23355, .T. ) ;
#27366=VECTOR ( 'NONE', #31642, 1000.000000000000000 ) ;
#27367=DIRECTION ( 'NONE',  ( 0.000000000000000000, 0.000000000000000000, 1.000000000000000000 ) ) ;
#27368=CARTESIAN_POINT ( 'NONE',  ( -7.100000000000013856, 12.50000000000000000, 3.702399969078682407 ) ) ;
#27370=DIRECTION ( 'NONE',  ( -4.274815082592931898E-19, -0.9999939076577903929, -0.003490651415223739937 ) ) ;
#27371=CIRCLE ( 'NONE', #79717, 0.06509327318403745899 ) ;
#27372=DIRECTION ( 'NONE',  ( 0.000000000000000000, -0.000000000000000000, 1.000000000000000000 ) ) ;
#27373=VERTEX_POINT ( 'NONE', #88904 ) ;
#27374=DIRECTION ( 'NONE',  ( -0.000000000000000000, -1.000000000000000000, -0.000000000000000000 ) ) ;
#27375=VERTEX_POINT ( 'NONE', #37239 ) ;
#27376=AXIS2_PLACEMENT_3D ( 'NONE', #20027, #38391, #355 ) ;
#27377=ORIENTED_EDGE ( 'NONE', *, *, #109507, .T. ) ;
#27378=FACE_OUTER_BOUND ( 'NONE', #78331, .T. ) ;
#27379=ORIENTED_EDGE ( 'NONE', *, *, #83031, .F. ) ;
#27380=CARTESIAN_POINT ( 'NONE',  ( 14.99999999999992895, 2.500000000000000000, -2.276824562219559311E-15 ) ) ;
#27381=FACE_BOUND ( 'NONE', #70810, .T. ) ;
#27382=ORIENTED_EDGE ( 'NONE', *, *, #94549, .F. ) ;
#27383=DIRECTION ( 'NONE',  ( 0.000000000000000000, 0.000000000000000000, -1.000000000000000000 ) ) ;
#27384=ORIENTED_EDGE ( 'NONE', *, *, #47813, .T. ) ;
#27385=FACE_OUTER_BOUND ( 'NONE', #40599, .T. ) ;
#27386=LINE ( 'NONE', #56212, #23641 ) ;
#27387=DIRECTION ( 'NONE',  ( 0.000000000000000000, 0.000000000000000000, 1.000000000000000000 ) ) ;
#27388=ADVANCED_FACE ( 'NONE', ( #8393 ), #74286, .T. ) ;
#27389=CARTESIAN_POINT ( 'NONE',  ( -7.900000000000014566, 2.500000000000000000, -2.276824562219559311E-15 ) ) ;
#27390=LINE ( 'NONE', #16908, #51667 ) ;
#27391=ORIENTED_EDGE ( 'NONE', *, *, #91843, .T. ) ;
#27392=ORIENTED_EDGE ( 'NONE', *, *, #85889, .F. ) ;
#27393=AXIS2_PLACEMENT_3D ( 'NONE', #509, #80389, #119644 ) ;
#27394=FACE_OUTER_BOUND ( 'NONE', #72156, .T. ) ;
#27395=DIRECTION ( 'NONE',  ( 0.000000000000000000, 0.000000000000000000, 1.000000000000000000 ) ) ;
#27396=CARTESIAN_POINT ( 'NONE',  ( 4.349999999999941025, 2.500000000000000000, -6.148780366869526226 ) ) ;
#27397=EDGE_CURVE ( 'NONE', #122201, #12963, #34592, .T. ) ;
#27398=ORIENTED_EDGE ( 'NONE', *, *, #122605, .T. ) ;
#27399=VERTEX_POINT ( 'NONE', #98701 ) ;
#27400=ORIENTED_EDGE ( 'NONE', *, *, #31111, .T. ) ;
#27401=ADVANCED_FACE ( 'NONE', ( #57516 ), #126512, .T. ) ;
#27402=DIRECTION ( 'NONE',  ( 0.000000000000000000, 0.000000000000000000, -1.000000000000000000 ) ) ;
#27403=EDGE_CURVE ( 'NONE', #3522, #110270, #59641, .T. ) ;
#27404=VECTOR ( 'NONE', #53700, 1000.000000000000000 ) ;
#27405=DIRECTION ( 'NONE',  ( 0.000000000000000000, 0.000000000000000000, -1.000000000000000000 ) ) ;
#27406=AXIS2_PLACEMENT_3D ( 'NONE', #16782, #15509, #76386 ) ;
#27407=CARTESIAN_POINT ( 'NONE',  ( 3.149999999999944400, 12.50000000000000000, 2.511473670974873507 ) ) ;
#27408=ADVANCED_FACE ( 'NONE', ( #9039 ), #48997, .T. ) ;
#27410=CARTESIAN_POINT ( 'NONE',  ( -3.350000000000029399, 12.50000000000000000, 6.495190528383297135 ) ) ;
#27411=LINE ( 'NONE', #35966, #91994 ) ;
#27412=CARTESIAN_POINT ( 'NONE',  ( 11.64999999999990621, 2.500000000000000000, -2.165063509461101710 ) ) ;
#27413=DIRECTION ( 'NONE',  ( 0.000000000000000000, 0.000000000000000000, -1.000000000000000000 ) ) ;
#27414=DIRECTION ( 'NONE',  ( 0.000000000000000000, 0.000000000000000000, 1.000000000000000000 ) ) ;
#27416=EDGE_CURVE ( 'NONE', #104801, #33641, #47698, .T. ) ;
#27418=EDGE_CURVE ( 'NONE', #16543, #80247, #91003, .T. ) ;
#27419=EDGE_LOOP ( 'NONE', ( #52545, #104144 ) ) ;
#27420=AXIS2_PLACEMENT_3D ( 'NONE', #56410, #115303, #6013 ) ;
#27421=EDGE_CURVE ( 'NONE', #75945, #17249, #107727, .T. ) ;
#27422=ORIENTED_EDGE ( 'NONE', *, *, #13004, .F. ) ;
#27423=EDGE_CURVE ( 'NONE', #99834, #70878, #57564, .T. ) ;
#27424=DIRECTION ( 'NONE',  ( 0.000000000000000000, 1.000000000000000000, 0.000000000000000000 ) ) ;
#27425=ORIENTED_EDGE ( 'NONE', *, *, #42959, .F. ) ;
#27426=ORIENTED_EDGE ( 'NONE', *, *, #37422, .T. ) ;
#27427=CARTESIAN_POINT ( 'NONE',  ( 9.999999999999914735, 2.500000000000000000, 0.6928203230275494784 ) ) ;
#27428=CARTESIAN_POINT ( 'NONE',  ( 8.749999999999923617, 12.50000000000000000, 1.472243186433545459 ) ) ;
#27429=CARTESIAN_POINT ( 'NONE',  ( -6.900000000000019007, 2.500000000000000000, 0.2464101615137735679 ) ) ;
#27430=ADVANCED_FACE ( 'NONE', ( #18214 ), #61779, .T. ) ;
#27431=AXIS2_PLACEMENT_3D ( 'NONE', #48919, #38458, #88823 ) ;
#27432=DIRECTION ( 'NONE',  ( -0.000000000000000000, -1.000000000000000000, -0.000000000000000000 ) ) ;
#27434=DIRECTION ( 'NONE',  ( -4.274815082592931898E-19, -0.9999939076577903929, -0.003490651415223739937 ) ) ;
#27435=CARTESIAN_POINT ( 'NONE',  ( 10.84999999999991260, 2.500000000000000000, -2.165063509461101710 ) ) ;
#27436=EDGE_LOOP ( 'NONE', ( #36660, #54335 ) ) ;
#27437=DIRECTION ( 'NONE',  ( -0.000000000000000000, 1.000000000000000000, -0.000000000000000000 ) ) ;
#27438=VECTOR ( 'NONE', #92718, 1000.000000000000000 ) ;
#27439=CARTESIAN_POINT ( 'NONE',  ( -14.54999999999998472, 2.500000000000000000, -2.265063509461099578 ) ) ;
#27440=ORIENTED_EDGE ( 'NONE', *, *, #77326, .T. ) ;
#27441=CONICAL_SURFACE ( 'NONE', #98538, 0.09999999999999982514, 0.003490658503988666988 ) ;
#27442=AXIS2_PLACEMENT_3D ( 'NONE', #5046, #92814, #54790 ) ;
#27443=ORIENTED_EDGE ( 'NONE', *, *, #104376, .F. ) ;
#27444=VERTEX_POINT ( 'NONE', #60108 ) ;
#27445=VERTEX_POINT ( 'NONE', #100016 ) ;
#27446=CARTESIAN_POINT ( 'NONE',  ( -8.550000000000011369, 2.500000000000000000, -2.411473670974877859 ) ) ;
#27447=PLANE ( 'NONE',  #47841 ) ;
#27448=EDGE_LOOP ( 'NONE', ( #90648, #79390 ) ) ;
#27449=FACE_OUTER_BOUND ( 'NONE', #14203, .T. ) ;
#27450=DIRECTION ( 'NONE',  ( -0.000000000000000000, -1.000000000000000000, -0.000000000000000000 ) ) ;
#27451=FACE_OUTER_BOUND ( 'NONE', #94560, .T. ) ;
#27452=ORIENTED_EDGE ( 'NONE', *, *, #101717, .F. ) ;
#27453=DIRECTION ( 'NONE',  ( 0.000000000000000000, 0.000000000000000000, 1.000000000000000000 ) ) ;
#27454=CARTESIAN_POINT ( 'NONE',  ( 7.299999999999926104, 2.500000000000000000, 4.776537180435972196 ) ) ;
#27455=ORIENTED_EDGE ( 'NONE', *, *, #125149, .T. ) ;
#27456=EDGE_CURVE ( 'NONE', #44454, #6764, #118190, .T. ) ;
#27457=VERTEX_POINT ( 'NONE', #98069 ) ;
#27458=VERTEX_POINT ( 'NONE', #48333 ) ;
#27459=AXIS2_PLACEMENT_3D ( 'NONE', #65263, #105199, #120190 ) ;
#27460=DIRECTION ( 'NONE',  ( 0.000000000000000000, 0.000000000000000000, 1.000000000000000000 ) ) ;
#27461=AXIS2_PLACEMENT_3D ( 'NONE', #115463, #46110, #125942 ) ;
#27462=FACE_OUTER_BOUND ( 'NONE', #106268, .T. ) ;
#27463=AXIS2_PLACEMENT_3D ( 'NONE', #76446, #125533, #14906 ) ;
#27464=VECTOR ( 'NONE', #117535, 1000.000000000000000 ) ;
#27465=CIRCLE ( 'NONE', #71304, 0.06509327318403745899 ) ;
#27466=ORIENTED_EDGE ( 'NONE', *, *, #16617, .T. ) ;
#27467=CARTESIAN_POINT ( 'NONE',  ( 1.849999999999950129, 2.500000000000000000, -6.941600689897078347 ) ) ;
#27468=DIRECTION ( 'NONE',  ( 0.000000000000000000, 0.000000000000000000, 1.000000000000000000 ) ) ;
#27469=ADVANCED_FACE ( 'NONE', ( #503 ), #19913, .T. ) ;
#27470=CARTESIAN_POINT ( 'NONE',  ( -1.650000000000034328, 2.500000000000000000, -6.495190528383302464 ) ) ;
#27472=EDGE_LOOP ( 'NONE', ( #9671, #79832 ) ) ;
#27473=DIRECTION ( 'NONE',  ( 0.000000000000000000, 1.000000000000000000, 0.000000000000000000 ) ) ;
#27474=EDGE_LOOP ( 'NONE', ( #73415, #69415, #94859, #107857 ) ) ;
#27475=ORIENTED_EDGE ( 'NONE', *, *, #5844, .F. ) ;
#27476=DIRECTION ( 'NONE',  ( 0.000000000000000000, 1.000000000000000000, 0.000000000000000000 ) ) ;
#27477=ORIENTED_EDGE ( 'NONE', *, *, #24033, .F. ) ;
#27478=DIRECTION ( 'NONE',  ( 0.000000000000000000, 0.000000000000000000, 1.000000000000000000 ) ) ;
#27479=FACE_BOUND ( 'NONE', #63238, .T. ) ;
#27480=CARTESIAN_POINT ( 'NONE',  ( 17.49862860983209956, 2.500000000000000000, 4.081131818001135336 ) ) ;
#27482=FACE_OUTER_BOUND ( 'NONE', #7828, .T. ) ;
#27483=ORIENTED_EDGE ( 'NONE', *, *, #53407, .T. ) ;
#27484=DIRECTION ( 'NONE',  ( 0.000000000000000000, -0.9999939076577903929, 0.003490651415223739937 ) ) ;
#27485=CARTESIAN_POINT ( 'NONE',  ( -6.900000000000019007, 2.500000000000000000, -4.776537180435978414 ) ) ;
#27486=FACE_OUTER_BOUND ( 'NONE', #47532, .T. ) ;
#27487=DIRECTION ( 'NONE',  ( -0.000000000000000000, 1.000000000000000000, -0.000000000000000000 ) ) ;
#27488=ORIENTED_EDGE ( 'NONE', *, *, #118546, .T. ) ;
#27489=CIRCLE ( 'NONE', #48443, 0.09999999999999999167 ) ;
#27490=DIRECTION ( 'NONE',  ( 0.000000000000000000, 0.000000000000000000, -1.000000000000000000 ) ) ;
#27491=CONICAL_SURFACE ( 'NONE', #65144, 0.1000000000000002554, 0.003490658503988666988 ) ;
#27492=ADVANCED_FACE ( 'NONE', ( #101311 ), #92779, .T. ) ;
#27493=DIRECTION ( 'NONE',  ( 0.000000000000000000, -0.000000000000000000, 1.000000000000000000 ) ) ;
#27494=ORIENTED_EDGE ( 'NONE', *, *, #17297, .F. ) ;
#27495=DIRECTION ( 'NONE',  ( -0.000000000000000000, -1.000000000000000000, -0.000000000000000000 ) ) ;
#27496=LINE ( 'NONE', #67413, #86103 ) ;
#27497=FACE_BOUND ( 'NONE', #124312, .T. ) ;
#27498=AXIS2_PLACEMENT_3D ( 'NONE', #7840, #98155, #119099 ) ;
#27499=ADVANCED_FACE ( 'NONE', ( #52845 ), #68013, .T. ) ;
#27501=AXIS2_PLACEMENT_3D ( 'NONE', #46432, #26165, #114524 ) ;
#27502=ORIENTED_EDGE ( 'NONE', *, *, #19719, .F. ) ;
#27503=FACE_OUTER_BOUND ( 'NONE', #35120, .T. ) ;
#27504=EDGE_CURVE ( 'NONE', #72741, #19960, #11577, .T. ) ;
#27505=ORIENTED_EDGE ( 'NONE', *, *, #107523, .F. ) ;
#27506=EDGE_CURVE ( 'NONE', #63975, #95323, #52203, .T. ) ;
#27507=EDGE_LOOP ( 'NONE', ( #126625, #120140 ) ) ;
#27508=CARTESIAN_POINT ( 'NONE',  ( 18.29531403502779696, 0.5011766475904850804, -4.780851392375763176 ) ) ;
#27509=ADVANCED_FACE ( 'NONE', ( #103238 ), #38803, .T. ) ;
#27512=ADVANCED_FACE ( 'NONE', ( #1794 ), #23368, .T. ) ;
#27513=EDGE_LOOP ( 'NONE', ( #351, #67100 ) ) ;
#27514=AXIS2_PLACEMENT_3D ( 'NONE', #67739, #88002, #97840 ) ;
#27515=DIRECTION ( 'NONE',  ( 0.000000000000000000, 0.000000000000000000, 1.000000000000000000 ) ) ;
#27516=DIRECTION ( 'NONE',  ( -0.000000000000000000, -1.000000000000000000, -0.000000000000000000 ) ) ;
#27517=AXIS2_PLACEMENT_3D ( 'NONE', #84013, #104932, #55218 ) ;
#27518=VECTOR ( 'NONE', #69158, 1000.000000000000000 ) ;
#27519=FACE_OUTER_BOUND ( 'NONE', #111862, .T. ) ;
#27520=EDGE_CURVE ( 'NONE', #115678, #126433, #116038, .T. ) ;
#27521=VECTOR ( 'NONE', #21233, 1000.000000000000000 ) ;
#27522=EDGE_CURVE ( 'NONE', #114128, #102404, #84740, .T. ) ;
#27523=ADVANCED_FACE ( 'NONE', ( #51569 ), #13626, .T. ) ;
#27524=VERTEX_POINT ( 'NONE', #91475 ) ;
#27525=DIRECTION ( 'NONE',  ( -0.000000000000000000, -1.000000000000000000, -0.000000000000000000 ) ) ;
#27526=AXIS2_PLACEMENT_3D ( 'NONE', #107388, #79233, #9188 ) ;
#27527=CIRCLE ( 'NONE', #123674, 0.1000000000000002554 ) ;
#27528=CARTESIAN_POINT ( 'NONE',  ( 12.09999999999990195, 12.50000000000000000, -0.6928203230275541413 ) ) ;
#27529=DIRECTION ( 'NONE',  ( 0.000000000000000000, 0.000000000000000000, -1.000000000000000000 ) ) ;
#27530=DIRECTION ( 'NONE',  ( 0.000000000000000000, 1.000000000000000000, 0.000000000000000000 ) ) ;
#27531=EDGE_LOOP ( 'NONE', ( #62266, #43177, #118415, #85294 ) ) ;
#27532=DIRECTION ( 'NONE',  ( 0.000000000000000000, 0.000000000000000000, -1.000000000000000000 ) ) ;
#27533=VERTEX_POINT ( 'NONE', #112418 ) ;
#27534=DIRECTION ( 'NONE',  ( 0.000000000000000000, 0.000000000000000000, 1.000000000000000000 ) ) ;
#27535=ORIENTED_EDGE ( 'NONE', *, *, #80141, .F. ) ;
#27536=CARTESIAN_POINT ( 'NONE',  ( 8.099999999999921485, 2.500000000000000000, -0.3464101615137783474 ) ) ;
#27537=DIRECTION ( 'NONE',  ( 0.000000000000000000, 0.000000000000000000, 1.000000000000000000 ) ) ;
#27538=FACE_OUTER_BOUND ( 'NONE', #98138, .T. ) ;
#27539=DIRECTION ( 'NONE',  ( -0.000000000000000000, 1.000000000000000000, -0.000000000000000000 ) ) ;
#27540=ORIENTED_EDGE ( 'NONE', *, *, #9967, .F. ) ;
#27541=DIRECTION ( 'NONE',  ( 0.000000000000000000, 0.000000000000000000, 1.000000000000000000 ) ) ;
#27542=CARTESIAN_POINT ( 'NONE',  ( 5.849999999999933031, 2.500000000000000000, -1.472243186433550122 ) ) ;
#27543=DIRECTION ( 'NONE',  ( -0.000000000000000000, 1.000000000000000000, -0.000000000000000000 ) ) ;
#27544=CARTESIAN_POINT ( 'NONE',  ( -13.29999999999998828, 12.50000000000000000, 4.330127018922196314 ) ) ;
#27545=LINE ( 'NONE', #46550, #32797 ) ;
#27546=ORIENTED_EDGE ( 'NONE', *, *, #105170, .T. ) ;
#27547=ORIENTED_EDGE ( 'NONE', *, *, #70008, .T. ) ;
#27548=CARTESIAN_POINT ( 'NONE',  ( 2.049999999999950084, 2.500000000000000000, 2.065063509461097624 ) ) ;
#27549=ORIENTED_EDGE ( 'NONE', *, *, #25569, .T. ) ;
#27550=VECTOR ( 'NONE', #92218, 1000.000000000000000 ) ;
#27551=CARTESIAN_POINT ( 'NONE',  ( 8.949999999999917577, 12.50000000000000000, -2.576566944158915184 ) ) ;
#27552=AXIS2_PLACEMENT_3D ( 'NONE', #31188, #71093, #53393 ) ;
#27553=AXIS2_PLACEMENT_3D ( 'NONE', #102312, #50613, #70914 ) ;
#27554=ORIENTED_EDGE ( 'NONE', *, *, #4010, .F. ) ;
#27555=VERTEX_POINT ( 'NONE', #121570 ) ;
#27556=ORIENTED_EDGE ( 'NONE', *, *, #26531, .F. ) ;
#27557=FACE_OUTER_BOUND ( 'NONE', #50721, .T. ) ;
#27558=DIRECTION ( 'NONE',  ( 0.000000000000000000, 0.000000000000000000, -1.000000000000000000 ) ) ;
#27559=AXIS2_PLACEMENT_3D ( 'NONE', #62124, #3205, #102042 ) ;
#27560=CARTESIAN_POINT ( 'NONE',  ( 1.899999999999951283, 2.500000000000000000, -3.983716857408426293 ) ) ;
#27561=AXIS2_PLACEMENT_3D ( 'NONE', #1011, #122088, #92618 ) ;
#27562=CARTESIAN_POINT ( 'NONE',  ( 4.149999999999938183, 2.500000000000000000, 7.288010851410849256 ) ) ;
#27563=CARTESIAN_POINT ( 'NONE',  ( 5.799999999999934985, 12.50000000000000000, -4.330127018922201643 ) ) ;
#27564=AXIS2_PLACEMENT_3D ( 'NONE', #8865, #127379, #48826 ) ;
#27565=DIRECTION ( 'NONE',  ( 0.000000000000000000, -0.9999939076577903929, 0.003490651415223739937 ) ) ;
#27566=CARTESIAN_POINT ( 'NONE',  ( 9.399999999999918643, 2.500000000000000000, 0.2464101615137736789 ) ) ;
#27567=CIRCLE ( 'NONE', #25511, 0.1000000000000002554 ) ;
#27568=VERTEX_POINT ( 'NONE', #43057 ) ;
#27569=EDGE_CURVE ( 'NONE', #69598, #3939, #40860, .T. ) ;
#27570=DIRECTION ( 'NONE',  ( 0.000000000000000000, 0.000000000000000000, -1.000000000000000000 ) ) ;
#27571=VERTEX_POINT ( 'NONE', #53499 ) ;
#27572=ADVANCED_FACE ( 'NONE', ( #102577 ), #82958, .T. ) ;
#27573=ORIENTED_EDGE ( 'NONE', *, *, #36673, .T. ) ;
#27574=EDGE_LOOP ( 'NONE', ( #49679, #99683 ) ) ;
#27575=ORIENTED_EDGE ( 'NONE', *, *, #6966, .F. ) ;
#27577=CARTESIAN_POINT ( 'NONE',  ( 8.949999999999921130, 2.500000000000000000, 1.818653347947321475 ) ) ;
#27578=EDGE_LOOP ( 'NONE', ( #96925, #37069, #119605, #49308 ) ) ;
#27579=ORIENTED_EDGE ( 'NONE', *, *, #62145, .T. ) ;
#27580=ADVANCED_FACE ( 'NONE', ( #110470 ), #69237, .T. ) ;
#27581=CARTESIAN_POINT ( 'NONE',  ( 3.099999999999944134, 2.500000000000000000, 4.776537180435972196 ) ) ;
#27582=DIRECTION ( 'NONE',  ( 0.000000000000000000, 0.000000000000000000, 1.000000000000000000 ) ) ;
#27583=FACE_OUTER_BOUND ( 'NONE', #111169, .T. ) ;
#27584=CARTESIAN_POINT ( 'NONE',  ( 3.099999999999943245, 12.50000000000000000, 3.983716857408420076 ) ) ;
#27585=DIRECTION ( 'NONE',  ( 0.000000000000000000, -0.9999939076577903929, 0.003490651415223739937 ) ) ;
#27586=EDGE_LOOP ( 'NONE', ( #97878, #43452 ) ) ;
#27587=CARTESIAN_POINT ( 'NONE',  ( 6.849999999999930367, 2.500000000000000000, -6.841600689897078702 ) ) ;
#27588=AXIS2_PLACEMENT_3D ( 'NONE', #82214, #24576, #112321 ) ;
#27589=ORIENTED_EDGE ( 'NONE', *, *, #48211, .F. ) ;
#27590=CARTESIAN_POINT ( 'NONE',  ( -14.34999999999998543, 2.500000000000000000, 1.718653347947325383 ) ) ;
#27591=EDGE_LOOP ( 'NONE', ( #73719, #118625 ) ) ;
#27592=CARTESIAN_POINT ( 'NONE',  ( -3.150000000000029665, 2.500000000000000000, 6.841600689897072485 ) ) ;
#27594=EDGE_CURVE ( 'NONE', #3622, #5490, #75498, .T. ) ;
#27595=ORIENTED_EDGE ( 'NONE', *, *, #101557, .T. ) ;
#27596=AXIS2_PLACEMENT_3D ( 'NONE', #71782, #30583, #50852 ) ;
#27597=FACE_OUTER_BOUND ( 'NONE', #117358, .T. ) ;
#27598=DIRECTION ( 'NONE',  ( 0.000000000000000000, 0.000000000000000000, 1.000000000000000000 ) ) ;
#27600=CARTESIAN_POINT ( 'NONE',  ( 8.949999999999917577, 2.500000000000000000, 6.048780366869520364 ) ) ;
#27601=CIRCLE ( 'NONE', #75625, 0.09999999999999982514 ) ;
#27602=CARTESIAN_POINT ( 'NONE',  ( -2.700000000000029932, 12.50000000000000000, -4.611443907251939756 ) ) ;
#27603=FACE_OUTER_BOUND ( 'NONE', #125930, .T. ) ;
#27604=ORIENTED_EDGE ( 'NONE', *, *, #80513, .T. ) ;
#27605=LINE ( 'NONE', #8604, #10092 ) ;
#27606=DIRECTION ( 'NONE',  ( 0.000000000000000000, 0.000000000000000000, 1.000000000000000000 ) ) ;
#27607=DIRECTION ( 'NONE',  ( -0.000000000000000000, 1.000000000000000000, -0.000000000000000000 ) ) ;
#27608=DIRECTION ( 'NONE',  ( -0.000000000000000000, 1.000000000000000000, -0.000000000000000000 ) ) ;
#27609=FACE_OUTER_BOUND ( 'NONE', #20181, .T. ) ;
#27610=ORIENTED_EDGE ( 'NONE', *, *, #91523, .F. ) ;
#27611=EDGE_CURVE ( 'NONE', #36319, #78931, #104837, .T. ) ;
#27612=AXIS2_PLACEMENT_3D ( 'NONE', #19808, #80007, #119939 ) ;
#27613=CIRCLE ( 'NONE', #100771, 0.06509327318403743123 ) ;
#27614=VECTOR ( 'NONE', #77950, 1000.000000000000000 ) ;
#27615=ORIENTED_EDGE ( 'NONE', *, *, #127563, .F. ) ;
#27616=DIRECTION ( 'NONE',  ( 0.000000000000000000, 0.000000000000000000, 1.000000000000000000 ) ) ;
#27617=CIRCLE ( 'NONE', #17133, 0.09999999999999999167 ) ;
#27618=EDGE_LOOP ( 'NONE', ( #33953, #103627 ) ) ;
#27619=CARTESIAN_POINT ( 'NONE',  ( -5.850000000000018296, 12.50000000000000000, 5.867463478539781896 ) ) ;
#27620=PLANE ( 'NONE',  #110787 ) ;
#27621=CONICAL_SURFACE ( 'NONE', #40265, 0.1000000000000000472, 0.003490658503988666988 ) ;
#27622=ORIENTED_EDGE ( 'NONE', *, *, #39223, .T. ) ;
#27624=CARTESIAN_POINT ( 'NONE',  ( 6.649999999999928413, 12.50000000000000000, 1.407149913249508000 ) ) ;
#27625=ADVANCED_FACE ( 'NONE', ( #33844 ), #111085, .T. ) ;
#27626=DIRECTION ( 'NONE',  ( 0.000000000000000000, 1.000000000000000000, 0.000000000000000000 ) ) ;
#27627=LINE ( 'NONE', #68857, #62311 ) ;
#27628=EDGE_LOOP ( 'NONE', ( #5244, #92038 ) ) ;
#27629=CARTESIAN_POINT ( 'NONE',  ( -3.100000000000028511, 12.50000000000000000, -0.3464101615137782364 ) ) ;
#27630=CARTESIAN_POINT ( 'NONE',  ( 6.649999999999931077, 2.500000000000000000, -6.595190528383302109 ) ) ;
#27631=ORIENTED_EDGE ( 'NONE', *, *, #87397, .T. ) ;
#27632=DIRECTION ( 'NONE',  ( -0.000000000000000000, -1.000000000000000000, -0.000000000000000000 ) ) ;
#27633=DIRECTION ( 'NONE',  ( -1.000000000000000000, -0.000000000000000000, -0.000000000000000000 ) ) ;
#27634=DIRECTION ( 'NONE',  ( -0.000000000000000000, -1.000000000000000000, -0.000000000000000000 ) ) ;
#27635=ORIENTED_EDGE ( 'NONE', *, *, #13341, .T. ) ;
#27636=DIRECTION ( 'NONE',  ( 0.000000000000000000, 0.000000000000000000, -1.000000000000000000 ) ) ;
#27637=VECTOR ( 'NONE', #118159, 1000.000000000000000 ) ;
#27638=AXIS2_PLACEMENT_3D ( 'NONE', #19095, #118611, #109440 ) ;
#27639=AXIS2_PLACEMENT_3D ( 'NONE', #24232, #62868, #14389 ) ;
#27640=ORIENTED_EDGE ( 'NONE', *, *, #110561, .T. ) ;
#27641=FACE_OUTER_BOUND ( 'NONE', #14437, .T. ) ;
#27642=DIRECTION ( 'NONE',  ( 0.000000000000000000, 1.000000000000000000, 0.000000000000000000 ) ) ;
#27643=DIRECTION ( 'NONE',  ( 0.000000000000000000, 0.000000000000000000, 1.000000000000000000 ) ) ;
#27644=VERTEX_POINT ( 'NONE', #85525 ) ;
#27645=VECTOR ( 'NONE', #114114, 1000.000000000000000 ) ;
#27646=CARTESIAN_POINT ( 'NONE',  ( -3.550000000000028244, 2.500000000000000000, -1.718653347947326049 ) ) ;
#27647=CONICAL_SURFACE ( 'NONE', #88186, 0.09999999999999982514, 0.003490658503988666988 ) ;
#27648=AXIS2_PLACEMENT_3D ( 'NONE', #20980, #60902, #12437 ) ;
#27649=EDGE_CURVE ( 'NONE', #7845, #27568, #6515, .T. ) ;
#27650=PLANE ( 'NONE',  #1510 ) ;
#27651=CIRCLE ( 'NONE', #88290, 0.1000000000000000472 ) ;
#27652=ORIENTED_EDGE ( 'NONE', *, *, #28334, .T. ) ;
#27653=AXIS2_PLACEMENT_3D ( 'NONE', #50296, #79749, #9724 ) ;
#27654=CARTESIAN_POINT ( 'NONE',  ( -6.650000000000015454, 2.500000000000000000, 7.088010851410848190 ) ) ;
#27655=ORIENTED_EDGE ( 'NONE', *, *, #94549, .T. ) ;
#27656=CIRCLE ( 'NONE', #23475, 0.06509327318403745899 ) ;
#27657=DIRECTION ( 'NONE',  ( -0.000000000000000000, -1.000000000000000000, -0.000000000000000000 ) ) ;
#27658=EDGE_CURVE ( 'NONE', #57054, #86890, #54135, .T. ) ;
#27659=ORIENTED_EDGE ( 'NONE', *, *, #61396, .T. ) ;
#27660=DIRECTION ( 'NONE',  ( 1.000000000000000000, 0.000000000000000000, 0.000000000000000000 ) ) ;
#27661=DIRECTION ( 'NONE',  ( -0.000000000000000000, -1.000000000000000000, -0.000000000000000000 ) ) ;
#27662=EDGE_CURVE ( 'NONE', #64421, #96425, #48415, .T. ) ;
#27663=VERTEX_POINT ( 'NONE', #84223 ) ;
#27664=ADVANCED_FACE ( 'NONE', ( #44307 ), #35158, .T. ) ;
#27665=VERTEX_POINT ( 'NONE', #26608 ) ;
#27666=EDGE_CURVE ( 'NONE', #108022, #24264, #50472, .T. ) ;
#27667=ADVANCED_FACE ( 'NONE', ( #95352 ), #106453, .T. ) ;
#27668=LINE ( 'NONE', #19128, #111540 ) ;
#27669=CARTESIAN_POINT ( 'NONE',  ( -5.650000000000019895, 2.500000000000000000, 1.718653347947321386 ) ) ;
#27670=ORIENTED_EDGE ( 'NONE', *, *, #501, .T. ) ;
#27672=DIRECTION ( 'NONE',  ( 0.000000000000000000, 0.000000000000000000, -1.000000000000000000 ) ) ;
#27673=CARTESIAN_POINT ( 'NONE',  ( -8.150000000000014566, 12.50000000000000000, -6.213873640053559022 ) ) ;
#27674=ADVANCED_FACE ( 'NONE', ( #115616 ), #96422, .T. ) ;
#27675=CARTESIAN_POINT ( 'NONE',  ( -4.150000000000025224, 2.500000000000000000, 5.802370205355744659 ) ) ;
#27676=LINE ( 'NONE', #67605, #777 ) ;
#27678=DIRECTION ( 'NONE',  ( 0.000000000000000000, -0.9999939076577903929, 0.003490651415223739937 ) ) ;
#27679=DIRECTION ( 'NONE',  ( -0.000000000000000000, -1.000000000000000000, -0.000000000000000000 ) ) ;
#27680=EDGE_CURVE ( 'NONE', #78540, #114240, #98569, .T. ) ;
#27681=CIRCLE ( 'NONE', #82075, 0.06509327318403745899 ) ;
#27682=EDGE_CURVE ( 'NONE', #96759, #62016, #113164, .T. ) ;
#27683=CIRCLE ( 'NONE', #31913, 0.06509327318403745899 ) ;
#27684=ADVANCED_FACE ( 'NONE', ( #56051 ), #121563, .T. ) ;
#27685=ORIENTED_EDGE ( 'NONE', *, *, #14093, .T. ) ;
#27686=VERTEX_POINT ( 'NONE', #6293 ) ;
#27687=EDGE_LOOP ( 'NONE', ( #112663, #21964, #18805, #93427 ) ) ;
#27688=ORIENTED_EDGE ( 'NONE', *, *, #92306, .F. ) ;
#27689=DIRECTION ( 'NONE',  ( -0.000000000000000000, 1.000000000000000000, -0.000000000000000000 ) ) ;
#27690=DIRECTION ( 'NONE',  ( -0.000000000000000000, 1.000000000000000000, -0.000000000000000000 ) ) ;
#27691=CARTESIAN_POINT ( 'NONE',  ( -10.84999999999999964, 2.500000000000000000, 2.857883832488649301 ) ) ;
#27692=VERTEX_POINT ( 'NONE', #14822 ) ;
#27693=FACE_BOUND ( 'NONE', #24734, .T. ) ;
#27694=EDGE_LOOP ( 'NONE', ( #24589, #36246 ) ) ;
#27695=AXIS2_PLACEMENT_3D ( 'NONE', #67752, #88685, #9481 ) ;
#27696=ADVANCED_FACE ( 'NONE', ( #103881 ), #4474, .T. ) ;
#27697=CARTESIAN_POINT ( 'NONE',  ( -11.24999999999996270, 2.500000000000000000, 6.495190528383297135 ) ) ;
#27698=FACE_OUTER_BOUND ( 'NONE', #68940, .T. ) ;
#27699=AXIS2_PLACEMENT_3D ( 'NONE', #67013, #107605, #108874 ) ;
#27700=CIRCLE ( 'NONE', #92461, 0.1000000000000002554 ) ;
#27701=DIRECTION ( 'NONE',  ( 0.000000000000000000, 0.000000000000000000, 1.000000000000000000 ) ) ;
#27702=CIRCLE ( 'NONE', #92463, 0.06509327318403745899 ) ;
#27703=CARTESIAN_POINT ( 'NONE',  ( 0.7999999999999612976, 2.500000000000000000, 0.09999999999999989453 ) ) ;
#27704=DIRECTION ( 'NONE',  ( 0.000000000000000000, -0.000000000000000000, 1.000000000000000000 ) ) ;
#27705=DIRECTION ( 'NONE',  ( 0.000000000000000000, 0.000000000000000000, 1.000000000000000000 ) ) ;
#27706=CARTESIAN_POINT ( 'NONE',  ( -1.250000000000001110, 12.50000000000000000, -2.165063509461101710 ) ) ;
#27707=CARTESIAN_POINT ( 'NONE',  ( 0.4499999999999552136, 12.50000000000000000, 6.560283801567334372 ) ) ;
#27708=LINE ( 'NONE', #127225, #108024 ) ;
#27709=CONICAL_SURFACE ( 'NONE', #13122, 0.09999999999999982514, 0.003490658503988666988 ) ;
#27710=CARTESIAN_POINT ( 'NONE',  ( -4.350000000000027178, 12.50000000000000000, -6.213873640053564351 ) ) ;
#27711=CONICAL_SURFACE ( 'NONE', #15176, 0.1000000000000000472, 0.003490658503988666988 ) ;
#27712=EDGE_LOOP ( 'NONE', ( #4695, #127793 ) ) ;
#27713=ORIENTED_EDGE ( 'NONE', *, *, #127009, .T. ) ;
#27714=EDGE_LOOP ( 'NONE', ( #90110, #101518 ) ) ;
#27715=CIRCLE ( 'NONE', #2564, 0.09999999999999982514 ) ;
#27716=EDGE_LOOP ( 'NONE', ( #29334, #71069 ) ) ;
#27717=VECTOR ( 'NONE', #28245, 1000.000000000000000 ) ;
#27718=AXIS2_PLACEMENT_3D ( 'NONE', #90999, #52359, #81184 ) ;
#27719=FACE_OUTER_BOUND ( 'NONE', #13151, .T. ) ;
#27720=DIRECTION ( 'NONE',  ( 0.000000000000000000, 0.000000000000000000, 1.000000000000000000 ) ) ;
#27721=EDGE_LOOP ( 'NONE', ( #125055, #8708, #118166, #58505 ) ) ;
#27722=ORIENTED_EDGE ( 'NONE', *, *, #2526, .F. ) ;
#27723=EDGE_LOOP ( 'NONE', ( #9066, #22023, #50835, #42742 ) ) ;
#27724=CIRCLE ( 'NONE', #92574, 0.06509327318403745899 ) ;
#27725=CARTESIAN_POINT ( 'NONE',  ( 0.8499999999999553468, 2.500000000000000000, 2.165063509461097713 ) ) ;
#27726=AXIS2_PLACEMENT_3D ( 'NONE', #88371, #128342, #38677 ) ;
#27727=DIRECTION ( 'NONE',  ( 0.000000000000000000, 0.000000000000000000, 1.000000000000000000 ) ) ;
#27728=CARTESIAN_POINT ( 'NONE',  ( -4.150000000000024336, 2.500000000000000000, 2.265063509461097357 ) ) ;
#27729=DIRECTION ( 'NONE',  ( 0.000000000000000000, -0.000000000000000000, 1.000000000000000000 ) ) ;
#27730=DIRECTION ( 'NONE',  ( 0.000000000000000000, 0.000000000000000000, -1.000000000000000000 ) ) ;
#27731=ORIENTED_EDGE ( 'NONE', *, *, #117671, .F. ) ;
#27732=PLANE ( 'NONE',  #53794 ) ;
#27733=ORIENTED_EDGE ( 'NONE', *, *, #418, .T. ) ;
#27734=ADVANCED_FACE ( 'NONE', ( #64593 ), #73451, .T. ) ;
#27735=ORIENTED_EDGE ( 'NONE', *, *, #46467, .F. ) ;
#27737=ADVANCED_FACE ( 'NONE', ( #94693 ), #46264, .T. ) ;
#27738=DIRECTION ( 'NONE',  ( 0.000000000000000000, 0.000000000000000000, 1.000000000000000000 ) ) ;
#27739=CIRCLE ( 'NONE', #117599, 0.1000000000000002554 ) ;
#27740=ORIENTED_EDGE ( 'NONE', *, *, #33768, .T. ) ;
#27741=ORIENTED_EDGE ( 'NONE', *, *, #89105, .F. ) ;
#27742=CARTESIAN_POINT ( 'NONE',  ( 10.84999999999991260, 2.500000000000000000, -2.857883832488653741 ) ) ;
#27743=EDGE_CURVE ( 'NONE', #50291, #40749, #94380, .T. ) ;
#27744=DIRECTION ( 'NONE',  ( -0.000000000000000000, 1.000000000000000000, -0.000000000000000000 ) ) ;
#27745=CARTESIAN_POINT ( 'NONE',  ( -10.45000000000000462, 2.500000000000000000, -2.165063509461097713 ) ) ;
#27746=AXIS2_PLACEMENT_3D ( 'NONE', #121376, #103024, #111563 ) ;
#27747=DIRECTION ( 'NONE',  ( 0.000000000000000000, 1.000000000000000000, 0.000000000000000000 ) ) ;
#27748=CONICAL_SURFACE ( 'NONE', #77919, 0.09999999999999982514, 0.003490658503988666988 ) ;
#27749=AXIS2_PLACEMENT_3D ( 'NONE', #92981, #113909, #44507 ) ;
#27750=CARTESIAN_POINT ( 'NONE',  ( -0.6500000000000398792, 2.500000000000000000, -2.611473670974877592 ) ) ;
#27751=EDGE_LOOP ( 'NONE', ( #75579, #102905, #94369, #56284 ) ) ;
#27752=LINE ( 'NONE', #57881, #53271 ) ;
#27753=AXIS2_PLACEMENT_3D ( 'NONE', #5853, #35343, #3933 ) ;
#27754=VERTEX_POINT ( 'NONE', #38382 ) ;
#27755=DIRECTION ( 'NONE',  ( 0.000000000000000000, 0.000000000000000000, 1.000000000000000000 ) ) ;
#27756=CONICAL_SURFACE ( 'NONE', #100907, 0.1000000000000000472, 0.003490658503988666988 ) ;
#27757=ORIENTED_EDGE ( 'NONE', *, *, #4358, .F. ) ;
#27759=CARTESIAN_POINT ( 'NONE',  ( 3.099999999999943245, 12.50000000000000000, 3.983716857408420076 ) ) ;
#27760=ORIENTED_EDGE ( 'NONE', *, *, #234, .T. ) ;
#27761=AXIS2_PLACEMENT_3D ( 'NONE', #70999, #110901, #68404 ) ;
#27762=DIRECTION ( 'NONE',  ( 0.000000000000000000, 1.000000000000000000, 0.000000000000000000 ) ) ;
#27763=AXIS2_PLACEMENT_3D ( 'NONE', #97771, #8092, #48041 ) ;
#27764=DIRECTION ( 'NONE',  ( -4.274815082592931898E-19, -0.9999939076577903929, -0.003490651415223739937 ) ) ;
#27765=ORIENTED_EDGE ( 'NONE', *, *, #71786, .F. ) ;
#27766=CONICAL_SURFACE ( 'NONE', #29837, 0.1000000000000002554, 0.003490658503988666988 ) ;
#27767=DIRECTION ( 'NONE',  ( -0.000000000000000000, -1.000000000000000000, -0.000000000000000000 ) ) ;
#27768=VERTEX_POINT ( 'NONE', #28548 ) ;
#27769=ORIENTED_EDGE ( 'NONE', *, *, #21176, .F. ) ;
#27770=FACE_OUTER_BOUND ( 'NONE', #95680, .T. ) ;
#27771=DIRECTION ( 'NONE',  ( 0.000000000000000000, 0.000000000000000000, 1.000000000000000000 ) ) ;
#27773=CARTESIAN_POINT ( 'NONE',  ( -6.650000000000014566, 12.50000000000000000, 2.230156782645134950 ) ) ;
#27774=CIRCLE ( 'NONE', #123917, 0.06509327318403745899 ) ;
#27775=EDGE_CURVE ( 'NONE', #19384, #33136, #280, .T. ) ;
#27776=FACE_OUTER_BOUND ( 'NONE', #44642, .T. ) ;
#27778=AXIS2_PLACEMENT_3D ( 'NONE', #70631, #41836, #82409 ) ;
#27779=VERTEX_POINT ( 'NONE', #86812 ) ;
#27780=AXIS2_PLACEMENT_3D ( 'NONE', #129302, #119437, #29786 ) ;
#27781=DIRECTION ( 'NONE',  ( 0.000000000000000000, 0.000000000000000000, -1.000000000000000000 ) ) ;
#27782=DIRECTION ( 'NONE',  ( -4.274815082592931898E-19, -0.9999939076577903929, -0.003490651415223739937 ) ) ;
#27783=AXIS2_PLACEMENT_3D ( 'NONE', #15781, #114627, #24966 ) ;
#27784=VERTEX_POINT ( 'NONE', #69100 ) ;
#27785=EDGE_CURVE ( 'NONE', #16781, #110736, #37952, .T. ) ;
#27786=FACE_OUTER_BOUND ( 'NONE', #114348, .T. ) ;
#27787=DIRECTION ( 'NONE',  ( 0.000000000000000000, -0.9999939076577903929, 0.003490651415223739937 ) ) ;
#27788=DIRECTION ( 'NONE',  ( 0.000000000000000000, 0.000000000000000000, 1.000000000000000000 ) ) ;
#27789=ADVANCED_FACE ( 'NONE', ( #67814 ), #71383, .T. ) ;
#27790=DIRECTION ( 'NONE',  ( 0.000000000000000000, 0.000000000000000000, 1.000000000000000000 ) ) ;
#27791=AXIS2_PLACEMENT_3D ( 'NONE', #90606, #10736, #24938 ) ;
#27792=CARTESIAN_POINT ( 'NONE',  ( 3.349999999999944578, 2.500000000000000000, -1.472243186433550122 ) ) ;
#27793=VECTOR ( 'NONE', #80420, 1000.000000000000000 ) ;
#27794=ORIENTED_EDGE ( 'NONE', *, *, #121081, .F. ) ;
#27795=VECTOR ( 'NONE', #8541, 1000.000000000000000 ) ;
#27796=VECTOR ( 'NONE', #116658, 1000.000000000000000 ) ;
#27797=DIRECTION ( 'NONE',  ( 0.000000000000000000, 0.000000000000000000, 1.000000000000000000 ) ) ;
#27798=CARTESIAN_POINT ( 'NONE',  ( -1.250000000000037970, 2.500000000000000000, 7.288010851410849256 ) ) ;
#27799=EDGE_CURVE ( 'NONE', #59725, #122166, #10733, .T. ) ;
#27800=CIRCLE ( 'NONE', #9019, 0.06509327318403745899 ) ;
#27801=ORIENTED_EDGE ( 'NONE', *, *, #91850, .F. ) ;
#27802=DIRECTION ( 'NONE',  ( 0.000000000000000000, 0.000000000000000000, 1.000000000000000000 ) ) ;
#27803=AXIS2_PLACEMENT_3D ( 'NONE', #18768, #47602, #96669 ) ;
#27804=VERTEX_POINT ( 'NONE', #56685 ) ;
#27805=CIRCLE ( 'NONE', #65362, 0.09999999999999982514 ) ;
#27806=AXIS2_PLACEMENT_3D ( 'NONE', #24222, #34710, #64138 ) ;
#27807=EDGE_LOOP ( 'NONE', ( #13982, #108014, #16873, #95720 ) ) ;
#27808=CONICAL_SURFACE ( 'NONE', #100977, 0.1000000000000002554, 0.003490658503988666988 ) ;
#27810=VECTOR ( 'NONE', #52809, 1000.000000000000000 ) ;
#27811=ORIENTED_EDGE ( 'NONE', *, *, #82925, .F. ) ;
#27812=DIRECTION ( 'NONE',  ( 0.000000000000000000, 1.000000000000000000, 0.000000000000000000 ) ) ;
#27813=CARTESIAN_POINT ( 'NONE',  ( 5.799999999999931433, 2.500000000000000000, 4.330127018922196314 ) ) ;
#27814=CARTESIAN_POINT ( 'NONE',  ( -7.900000000000011013, 2.500000000000000000, 3.537306695894645081 ) ) ;
#27815=VERTEX_POINT ( 'NONE', #107747 ) ;
#27816=CARTESIAN_POINT ( 'NONE',  ( -11.89999999999999503, 12.50000000000000000, 3.918623584224382839 ) ) ;
#27817=VECTOR ( 'NONE', #7733, 1000.000000000000000 ) ;
#27818=LINE ( 'NONE', #59243, #72444 ) ;
#27819=ORIENTED_EDGE ( 'NONE', *, *, #98033, .T. ) ;
#27820=DIRECTION ( 'NONE',  ( -4.274815082592931898E-19, -0.9999939076577903929, -0.003490651415223739937 ) ) ;
#27821=DIRECTION ( 'NONE',  ( 0.000000000000000000, 1.000000000000000000, 0.000000000000000000 ) ) ;
#27822=EDGE_LOOP ( 'NONE', ( #127485, #120002, #63055, #34759 ) ) ;
#27823=EDGE_CURVE ( 'NONE', #66532, #54360, #109688, .T. ) ;
#27824=ORIENTED_EDGE ( 'NONE', *, *, #56947, .T. ) ;
#27825=VERTEX_POINT ( 'NONE', #9553 ) ;
#27826=DIRECTION ( 'NONE',  ( 0.000000000000000000, 1.000000000000000000, 0.000000000000000000 ) ) ;
#27827=FACE_OUTER_BOUND ( 'NONE', #120210, .T. ) ;
#27828=CONICAL_SURFACE ( 'NONE', #121823, 0.1000000000000002554, 0.003490658503988666988 ) ;
#27829=DIRECTION ( 'NONE',  ( 0.000000000000000000, 0.000000000000000000, -1.000000000000000000 ) ) ;
#27830=CIRCLE ( 'NONE', #32065, 0.1000000000000002554 ) ;
#27831=EDGE_CURVE ( 'NONE', #53467, #96425, #37723, .T. ) ;
#27832=FACE_BOUND ( 'NONE', #76811, .T. ) ;
#27833=VERTEX_POINT ( 'NONE', #57357 ) ;
#27834=EDGE_CURVE ( 'NONE', #66455, #32421, #6936, .T. ) ;
#27835=CARTESIAN_POINT ( 'NONE',  ( -5.200000000000025935, 2.500000000000000000, -4.083716857408426826 ) ) ;
#27836=DIRECTION ( 'NONE',  ( 0.000000000000000000, 0.000000000000000000, 1.000000000000000000 ) ) ;
#27837=ORIENTED_EDGE ( 'NONE', *, *, #110569, .T. ) ;
#27838=VECTOR ( 'NONE', #23956, 1000.000000000000000 ) ;
#27839=CARTESIAN_POINT ( 'NONE',  ( -9.800000000000004263, 12.50000000000000000, 3.983716857408420076 ) ) ;
#27840=CIRCLE ( 'NONE', #59167, 0.09999999999999999167 ) ;
#27841=CONICAL_SURFACE ( 'NONE', #86323, 0.1000000000000002554, 0.003490658503988666988 ) ;
#27842=EDGE_CURVE ( 'NONE', #34384, #106414, #8678, .T. ) ;
#27843=DIRECTION ( 'NONE',  ( -0.000000000000000000, -1.000000000000000000, -0.000000000000000000 ) ) ;
#27844=AXIS2_PLACEMENT_3D ( 'NONE', #94572, #95238, #96494 ) ;
#27845=ADVANCED_FACE ( 'NONE', ( #118210 ), #108942, .T. ) ;
#27846=LINE ( 'NONE', #49446, #63296 ) ;
#27847=EDGE_CURVE ( 'NONE', #107859, #128878, #125669, .T. ) ;
#27848=PLANE ( 'NONE',  #101514 ) ;
#27849=DIRECTION ( 'NONE',  ( 0.000000000000000000, 0.000000000000000000, -1.000000000000000000 ) ) ;
#27850=VECTOR ( 'NONE', #29567, 1000.000000000000000 ) ;
#27851=CONICAL_SURFACE ( 'NONE', #59174, 0.09999999999999999167, 0.003490658503988666988 ) ;
#27852=VECTOR ( 'NONE', #12692, 1000.000000000000000 ) ;
#27853=EDGE_CURVE ( 'NONE', #96425, #64421, #119410, .T. ) ;
#27854=EDGE_LOOP ( 'NONE', ( #67558, #3818, #63685, #16098 ) ) ;
#27855=VERTEX_POINT ( 'NONE', #58013 ) ;
#27856=ORIENTED_EDGE ( 'NONE', *, *, #86034, .F. ) ;
#27857=VERTEX_POINT ( 'NONE', #8885 ) ;
#27858=CONICAL_SURFACE ( 'NONE', #40397, 0.09999999999999999167, 0.003490658503988666988 ) ;
#27859=EDGE_LOOP ( 'NONE', ( #59435, #3534, #18983, #101536 ) ) ;
#27860=LINE ( 'NONE', #18682, #119521 ) ;
#27861=CIRCLE ( 'NONE', #9080, 0.1000000000000002554 ) ;
#27862=LINE ( 'NONE', #67781, #2876 ) ;
#27863=EDGE_LOOP ( 'NONE', ( #83414, #16814 ) ) ;
#27864=ADVANCED_FACE ( 'NONE', ( #59317 ), #48841, .T. ) ;
#27865=FACE_BOUND ( 'NONE', #124201, .T. ) ;
#27866=ADVANCED_FACE ( 'NONE', ( #128712 ), #42262, .T. ) ;
#27867=CIRCLE ( 'NONE', #61322, 1.000000000000000888 ) ;
#27868=FACE_OUTER_BOUND ( 'NONE', #105802, .T. ) ;
#27869=DIRECTION ( 'NONE',  ( 0.000000000000000000, 0.000000000000000000, 1.000000000000000000 ) ) ;
#27870=DIRECTION ( 'NONE',  ( 0.000000000000000000, 1.000000000000000000, 0.000000000000000000 ) ) ;
#27871=DIRECTION ( 'NONE',  ( -0.000000000000000000, -1.000000000000000000, -0.000000000000000000 ) ) ;
#27872=FACE_OUTER_BOUND ( 'NONE', #16345, .T. ) ;
#27873=EDGE_LOOP ( 'NONE', ( #45179, #80593, #42641, #90364 ) ) ;
#27874=FACE_OUTER_BOUND ( 'NONE', #40802, .T. ) ;
#27875=VECTOR ( 'NONE', #54530, 1000.000000000000000 ) ;
#27876=ORIENTED_EDGE ( 'NONE', *, *, #92685, .F. ) ;
#27877=VERTEX_POINT ( 'NONE', #48182 ) ;
#27878=ORIENTED_EDGE ( 'NONE', *, *, #123662, .F. ) ;
#27879=CARTESIAN_POINT ( 'NONE',  ( -3.150000000000029221, 2.500000000000000000, 2.511473670974873507 ) ) ;
#27880=DIRECTION ( 'NONE',  ( 0.000000000000000000, 1.000000000000000000, 0.000000000000000000 ) ) ;
#27881=CARTESIAN_POINT ( 'NONE',  ( 17.50000000000000355, -2.500000000000000000, -4.040567763475364060 ) ) ;
#27882=ORIENTED_EDGE ( 'NONE', *, *, #15872, .F. ) ;
#27883=CARTESIAN_POINT ( 'NONE',  ( 12.06068301339517390, 1.499999999999871436, -8.632777000277979340 ) ) ;
#27884=AXIS2_PLACEMENT_3D ( 'NONE', #74222, #114776, #5460 ) ;
#27885=CIRCLE ( 'NONE', #44516, 0.09999999999999982514 ) ;
#27886=DIRECTION ( 'NONE',  ( 0.000000000000000000, -0.000000000000000000, 1.000000000000000000 ) ) ;
#27887=PLANE ( 'NONE',  #89249 ) ;
#27888=CARTESIAN_POINT ( 'NONE',  ( 11.24999999999990585, 12.50000000000000000, -5.867463478539787225 ) ) ;
#27889=DIRECTION ( 'NONE',  ( -4.274815082592931898E-19, -0.9999939076577903929, -0.003490651415223739937 ) ) ;
#27890=CARTESIAN_POINT ( 'NONE',  ( 9.599999999999914380, 12.50000000000000000, 5.022947341949748790 ) ) ;
#27891=CARTESIAN_POINT ( 'NONE',  ( 2.699999999999947331, 2.500000000000000000, -4.776537180435978414 ) ) ;
#27892=CONICAL_SURFACE ( 'NONE', #40439, 0.09999999999999982514, 0.003490658503988666988 ) ;
#27893=ORIENTED_EDGE ( 'NONE', *, *, #80873, .T. ) ;
#27894=DIRECTION ( 'NONE',  ( 0.000000000000000000, -0.000000000000000000, 1.000000000000000000 ) ) ;
#27895=AXIS2_PLACEMENT_3D ( 'NONE', #65911, #46272, #76393 ) ;
#27896=AXIS2_PLACEMENT_3D ( 'NONE', #120145, #10797, #11471 ) ;
#27897=VERTEX_POINT ( 'NONE', #88074 ) ;
#27898=CIRCLE ( 'NONE', #88522, 0.09999999999999982514 ) ;
#27899=EDGE_CURVE ( 'NONE', #124875, #68434, #128032, .T. ) ;
#27900=ORIENTED_EDGE ( 'NONE', *, *, #52508, .F. ) ;
#27901=DIRECTION ( 'NONE',  ( 0.000000000000000000, 0.000000000000000000, 1.000000000000000000 ) ) ;
#27902=EDGE_CURVE ( 'NONE', #30611, #107580, #111185, .T. ) ;
#27903=CARTESIAN_POINT ( 'NONE',  ( 2.499999999999948930, 2.500000000000000000, -0.7928203230275542301 ) ) ;
#27904=DIRECTION ( 'NONE',  ( 0.000000000000000000, 0.000000000000000000, 1.000000000000000000 ) ) ;
#27905=AXIS2_PLACEMENT_3D ( 'NONE', #56992, #9197, #77934 ) ;
#27906=ORIENTED_EDGE ( 'NONE', *, *, #126318, .F. ) ;
#27907=VERTEX_POINT ( 'NONE', #12113 ) ;
#27908=DIRECTION ( 'NONE',  ( 0.000000000000000000, 0.000000000000000000, 1.000000000000000000 ) ) ;
#27909=CARTESIAN_POINT ( 'NONE',  ( 8.749999999999921840, 2.500000000000000000, 2.857883832488649301 ) ) ;
#27910=AXIS2_PLACEMENT_3D ( 'NONE', #67028, #74942, #46123 ) ;
#27911=AXIS2_PLACEMENT_3D ( 'NONE', #9558, #8251, #89403 ) ;
#27912=DIRECTION ( 'NONE',  ( 0.000000000000000000, 0.000000000000000000, -1.000000000000000000 ) ) ;
#27913=ORIENTED_EDGE ( 'NONE', *, *, #53160, .F. ) ;
#27914=VERTEX_POINT ( 'NONE', #122724 ) ;
#27915=CARTESIAN_POINT ( 'NONE',  ( -6.249999999999981348, 2.500000000000000000, 6.395190528383296602 ) ) ;
#27916=AXIS2_PLACEMENT_3D ( 'NONE', #309, #8849, #19983 ) ;
#27917=EDGE_LOOP ( 'NONE', ( #87129, #42352, #10195, #106893, #18727, #107926, #37885, #57074, #95702, #18397, #103397, #25314 ) ) ;
#27918=CARTESIAN_POINT ( 'NONE',  ( 13.29999999999989946, 12.50000000000000000, -2.385244779468109755E-15 ) ) ;
#27920=ORIENTED_EDGE ( 'NONE', *, *, #94666, .T. ) ;
#27921=CARTESIAN_POINT ( 'NONE',  ( -5.800000000000018474, 2.500000000000000000, -0.1000000000000022815 ) ) ;
#27922=FACE_OUTER_BOUND ( 'NONE', #31127, .T. ) ;
#27923=DIRECTION ( 'NONE',  ( -0.000000000000000000, 1.000000000000000000, -0.000000000000000000 ) ) ;
#27924=CARTESIAN_POINT ( 'NONE',  ( 0.1999999999999627909, 12.50000000000000000, 0.4115034346978132529 ) ) ;
#27925=ORIENTED_EDGE ( 'NONE', *, *, #49430, .T. ) ;
#27926=DIRECTION ( 'NONE',  ( 0.000000000000000000, 0.000000000000000000, 1.000000000000000000 ) ) ;
#27927=ORIENTED_EDGE ( 'NONE', *, *, #118289, .T. ) ;
#27928=ORIENTED_EDGE ( 'NONE', *, *, #43933, .F. ) ;
#27929=CONICAL_SURFACE ( 'NONE', #103143, 0.1000000000000002554, 0.003490658503988666988 ) ;
#27930=AXIS2_PLACEMENT_3D ( 'NONE', #124953, #35295, #73917 ) ;
#27931=DIRECTION ( 'NONE',  ( -0.000000000000000000, -1.000000000000000000, -0.000000000000000000 ) ) ;
#27932=DIRECTION ( 'NONE',  ( 0.000000000000000000, 1.000000000000000000, 0.000000000000000000 ) ) ;
#27933=CARTESIAN_POINT ( 'NONE',  ( -8.950000000000009948, 2.500000000000000000, 2.511473670974873507 ) ) ;
#27934=CARTESIAN_POINT ( 'NONE',  ( 9.399999999999918643, 2.500000000000000000, -0.3464101615137782364 ) ) ;
#27935=CARTESIAN_POINT ( 'NONE',  ( -13.09999999999999254, 12.50000000000000000, 0.3464101615137777923 ) ) ;
#27936=DIRECTION ( 'NONE',  ( 0.000000000000000000, 0.000000000000000000, -1.000000000000000000 ) ) ;
#27937=EDGE_CURVE ( 'NONE', #127206, #115023, #48515, .T. ) ;
#27938=VECTOR ( 'NONE', #124581, 1000.000000000000000 ) ;
#27939=CIRCLE ( 'NONE', #17456, 0.06509327318403745899 ) ;
#27940=DIRECTION ( 'NONE',  ( 0.000000000000000000, -0.000000000000000000, 1.000000000000000000 ) ) ;
#27941=CARTESIAN_POINT ( 'NONE',  ( 14.34999999999989306, 2.500000000000000000, -1.818653347947326138 ) ) ;
#27942=CARTESIAN_POINT ( 'NONE',  ( -9.400000000000007461, 2.500000000000000000, -0.4464101615137783252 ) ) ;
#27943=AXIS2_PLACEMENT_3D ( 'NONE', #74432, #44975, #44312 ) ;
#27944=VECTOR ( 'NONE', #31030, 1000.000000000000000 ) ;
#27945=CARTESIAN_POINT ( 'NONE',  ( -7.950000000000016165, 2.500000000000000000, -6.395190528383296602 ) ) ;
#27946=EDGE_CURVE ( 'NONE', #92039, #14604, #58984, .T. ) ;
#27947=CONICAL_SURFACE ( 'NONE', #59271, 0.09999999999999982514, 0.003490658503988666988 ) ;
#27948=AXIS2_PLACEMENT_3D ( 'NONE', #102287, #112107, #11958 ) ;
#27949=AXIS2_PLACEMENT_3D ( 'NONE', #125249, #116705, #55226 ) ;
#27950=EDGE_LOOP ( 'NONE', ( #114044, #15891, #108855, #83638 ) ) ;
#27951=DIRECTION ( 'NONE',  ( 0.000000000000000000, 0.000000000000000000, 1.000000000000000000 ) ) ;
#27952=CIRCLE ( 'NONE', #753, 0.06509327318403745899 ) ;
#27953=ADVANCED_FACE ( 'NONE', ( #90018 ), #69328, .T. ) ;
#27954=DIRECTION ( 'NONE',  ( 0.000000000000000000, 0.000000000000000000, 1.000000000000000000 ) ) ;
#27955=DIRECTION ( 'NONE',  ( -4.274815082592931898E-19, -0.9999939076577903929, -0.003490651415223739937 ) ) ;
#27956=EDGE_CURVE ( 'NONE', #100972, #91293, #91326, .T. ) ;
#27957=CARTESIAN_POINT ( 'NONE',  ( -1.050000000000037348, 12.50000000000000000, -6.841600689897078702 ) ) ;
#27958=DIRECTION ( 'NONE',  ( -4.274815082592931898E-19, -0.9999939076577903929, -0.003490651415223739937 ) ) ;
#27959=ORIENTED_EDGE ( 'NONE', *, *, #116604, .T. ) ;
#27960=DIRECTION ( 'NONE',  ( 0.000000000000000000, 0.000000000000000000, 1.000000000000000000 ) ) ;
#27961=ADVANCED_FACE ( 'NONE', ( #71047 ), #92324, .T. ) ;
#27962=DIRECTION ( 'NONE',  ( 0.000000000000000000, 0.000000000000000000, 1.000000000000000000 ) ) ;
#27963=CARTESIAN_POINT ( 'NONE',  ( -4.350000000000027178, 2.500000000000000000, -6.741600689897077281 ) ) ;
#27964=ORIENTED_EDGE ( 'NONE', *, *, #76774, .F. ) ;
#27965=ADVANCED_FACE ( 'NONE', ( #59968 ), #35898, .T. ) ;
#27966=AXIS2_PLACEMENT_3D ( 'NONE', #75316, #55036, #17002 ) ;
#27967=ORIENTED_EDGE ( 'NONE', *, *, #129400, .F. ) ;
#27969=ORIENTED_EDGE ( 'NONE', *, *, #90793, .T. ) ;
#27970=EDGE_LOOP ( 'NONE', ( #46516, #117415 ) ) ;
#27971=DIRECTION ( 'NONE',  ( 0.000000000000000000, 1.000000000000000000, 0.000000000000000000 ) ) ;
#27973=DIRECTION ( 'NONE',  ( -0.000000000000000000, -1.000000000000000000, -0.000000000000000000 ) ) ;
#27974=CARTESIAN_POINT ( 'NONE',  ( 0.8499999999999557909, 2.500000000000000000, -7.188010851410854052 ) ) ;
#27975=AXIS2_PLACEMENT_3D ( 'NONE', #4644, #54413, #74706 ) ;
#27976=CARTESIAN_POINT ( 'NONE',  ( -7.950000000000012612, 12.50000000000000000, 2.099970236277060032 ) ) ;
#27977=CONICAL_SURFACE ( 'NONE', #115701, 0.1000000000000002554, 0.003490658503988666988 ) ;
#27978=ORIENTED_EDGE ( 'NONE', *, *, #41327, .T. ) ;
#27979=DIRECTION ( 'NONE',  ( 0.000000000000000000, 0.000000000000000000, 1.000000000000000000 ) ) ;
#27980=ORIENTED_EDGE ( 'NONE', *, *, #122057, .F. ) ;
#27981=CARTESIAN_POINT ( 'NONE',  ( 87.50000000000001421, -3.974992050023849810, -6.359987280038161828 ) ) ;
#27982=CARTESIAN_POINT ( 'NONE',  ( 1.849999999999949685, 2.500000000000000000, -2.611473670974877592 ) ) ;
#27983=CARTESIAN_POINT ( 'NONE',  ( 20.64614705759265689, 2.669560853936145950, 2.247897417617497062 ) ) ;
#27984=DIRECTION ( 'NONE',  ( -0.000000000000000000, -1.000000000000000000, -0.000000000000000000 ) ) ;
#27985=DIRECTION ( 'NONE',  ( -0.000000000000000000, 1.000000000000000000, -0.000000000000000000 ) ) ;
#27986=AXIS2_PLACEMENT_3D ( 'NONE', #32475, #65102, #35669 ) ;
#27987=VECTOR ( 'NONE', #100493, 1000.000000000000000 ) ;
#27988=VERTEX_POINT ( 'NONE', #61886 ) ;
#27989=EDGE_CURVE ( 'NONE', #14553, #120064, #10831, .T. ) ;
#27990=ORIENTED_EDGE ( 'NONE', *, *, #53282, .T. ) ;
#27991=ORIENTED_EDGE ( 'NONE', *, *, #21194, .F. ) ;
#27992=EDGE_LOOP ( 'NONE', ( #104586, #83795, #77190, #39847 ) ) ;
#27993=FACE_OUTER_BOUND ( 'NONE', #61070, .T. ) ;
#27994=CARTESIAN_POINT ( 'NONE',  ( -0.8500000000000395017, 2.500000000000000000, 2.265063509461097357 ) ) ;
#27995=CARTESIAN_POINT ( 'NONE',  ( 7.949999999999922018, 12.50000000000000000, -2.099970236277064473 ) ) ;
#27996=ADVANCED_FACE ( 'NONE', ( #350 ), #71482, .T. ) ;
#27997=FACE_BOUND ( 'NONE', #116922, .T. ) ;
#27998=AXIS2_PLACEMENT_3D ( 'NONE', #108371, #18698, #98532 ) ;
#27999=LINE ( 'NONE', #99324, #47328 ) ;
#28000=DIRECTION ( 'NONE',  ( 0.000000000000000000, 0.000000000000000000, -1.000000000000000000 ) ) ;
#28001=ADVANCED_FACE ( 'NONE', ( #110323 ), #56797, .T. ) ;
#28002=DIRECTION ( 'NONE',  ( 0.000000000000000000, 1.000000000000000000, 0.000000000000000000 ) ) ;
#28003=CARTESIAN_POINT ( 'NONE',  ( -3.350000000000028955, 2.500000000000000000, 2.265063509461097357 ) ) ;
#28004=AXIS2_PLACEMENT_3D ( 'NONE', #7, #39951, #97565 ) ;
#28005=EDGE_CURVE ( 'NONE', #110872, #117851, #109036, .T. ) ;
#28007=EDGE_CURVE ( 'NONE', #34238, #49883, #54754, .T. ) ;
#28008=DIRECTION ( 'NONE',  ( 0.000000000000000000, 0.000000000000000000, 1.000000000000000000 ) ) ;
#28009=CONICAL_SURFACE ( 'NONE', #30084, 0.09999999999999982514, 0.003490658503988666988 ) ;
#28010=ADVANCED_FACE ( 'NONE', ( #60601 ), #110946, .T. ) ;
#28011=CARTESIAN_POINT ( 'NONE',  ( 10.64999999999991331, 2.500000000000000000, 6.841600689897072485 ) ) ;
#28012=EDGE_CURVE ( 'NONE', #16978, #109486, #23358, .T. ) ;
#28013=AXIS2_PLACEMENT_3D ( 'NONE', #16555, #66945, #118636 ) ;
#28014=CARTESIAN_POINT ( 'NONE',  ( 1.849999999999951017, 12.50000000000000000, -6.148780366869526226 ) ) ;
#28015=ADVANCED_FACE ( 'NONE', ( #90680 ), #17079, .T. ) ;
#28016=ORIENTED_EDGE ( 'NONE', *, *, #80704, .F. ) ;
#28017=ORIENTED_EDGE ( 'NONE', *, *, #64941, .T. ) ;
#28018=EDGE_LOOP ( 'NONE', ( #126773, #106678, #55837, #23995 ) ) ;
#28019=EDGE_LOOP ( 'NONE', ( #37687, #68687, #106413, #62644 ) ) ;
#28020=PLANE ( 'NONE',  #61184 ) ;
#28021=FACE_BOUND ( 'NONE', #107538, .T. ) ;
#28023=DIRECTION ( 'NONE',  ( 0.000000000000000000, 0.000000000000000000, 1.000000000000000000 ) ) ;
#28024=EDGE_CURVE ( 'NONE', #40294, #108133, #82158, .T. ) ;
#28025=CONICAL_SURFACE ( 'NONE', #95215, 0.1000000000000000472, 0.003490658503988666988 ) ;
#28026=ORIENTED_EDGE ( 'NONE', *, *, #110170, .F. ) ;
#28027=LINE ( 'NONE', #17542, #128304 ) ;
#28028=AXIS2_PLACEMENT_3D ( 'NONE', #13692, #5162, #64733 ) ;
#28029=CARTESIAN_POINT ( 'NONE',  ( -7.100000000000017408, 2.500000000000000000, 0.6928203230275494784 ) ) ;
#28030=FACE_OUTER_BOUND ( 'NONE', #103751, .T. ) ;
#28031=EDGE_LOOP ( 'NONE', ( #72835, #59200 ) ) ;
#28032=CARTESIAN_POINT ( 'NONE',  ( -4.800000000000028244, 12.50000000000000000, -3.918623584224389056 ) ) ;
#28033=CARTESIAN_POINT ( 'NONE',  ( 5.649999999999934630, 2.500000000000000000, -1.918653347947325782 ) ) ;
#28034=VECTOR ( 'NONE', #23807, 1000.000000000000000 ) ;
#28035=CIRCLE ( 'NONE', #82433, 0.1000000000000002554 ) ;
#28036=AXIS2_PLACEMENT_3D ( 'NONE', #99127, #89296, #129255 ) ;
#28037=AXIS2_PLACEMENT_3D ( 'NONE', #118213, #99229, #59975 ) ;
#28038=ORIENTED_EDGE ( 'NONE', *, *, #60524, .F. ) ;
#28039=ORIENTED_EDGE ( 'NONE', *, *, #72789, .F. ) ;
#28040=FACE_OUTER_BOUND ( 'NONE', #56397, .T. ) ;
#28041=DIRECTION ( 'NONE',  ( 0.000000000000000000, 1.000000000000000000, 0.000000000000000000 ) ) ;
#28042=AXIS2_PLACEMENT_3D ( 'NONE', #77859, #106679, #128281 ) ;
#28043=AXIS2_PLACEMENT_3D ( 'NONE', #77916, #127666, #49134 ) ;
#28044=CARTESIAN_POINT ( 'NONE',  ( -12.89999999999999325, 12.50000000000000000, 0.7579135962115910452 ) ) ;
#28045=DIRECTION ( 'NONE',  ( 0.000000000000000000, 0.000000000000000000, 1.000000000000000000 ) ) ;
#28046=VERTEX_POINT ( 'NONE', #101154 ) ;
#28047=CARTESIAN_POINT ( 'NONE',  ( 9.999999999999912959, 12.50000000000000000, 3.637306695894644726 ) ) ;
#28048=VECTOR ( 'NONE', #113097, 1000.000000000000000 ) ;
#28049=EDGE_LOOP ( 'NONE', ( #74921, #99021, #73423, #31811 ) ) ;
#28050=ORIENTED_EDGE ( 'NONE', *, *, #113067, .T. ) ;
#28051=DIRECTION ( 'NONE',  ( 0.000000000000000000, 0.000000000000000000, 1.000000000000000000 ) ) ;
#28052=ORIENTED_EDGE ( 'NONE', *, *, #90273, .T. ) ;
#28053=DIRECTION ( 'NONE',  ( 0.000000000000000000, 1.000000000000000000, 0.000000000000000000 ) ) ;
#28054=FACE_BOUND ( 'NONE', #87674, .T. ) ;
#28055=ORIENTED_EDGE ( 'NONE', *, *, #116787, .T. ) ;
#28056=EDGE_CURVE ( 'NONE', #68041, #121003, #11474, .T. ) ;
#28057=DIRECTION ( 'NONE',  ( 0.000000000000000000, 0.000000000000000000, 1.000000000000000000 ) ) ;
#28058=EDGE_LOOP ( 'NONE', ( #124245, #129578, #58225, #39817 ) ) ;
#28059=CARTESIAN_POINT ( 'NONE',  ( -7.500000000000001776, 1.500000000000000000, 1.734723475976807094E-15 ) ) ;
#28060=CARTESIAN_POINT ( 'NONE',  ( 5.599999999999931255, 2.500000000000000000, 4.776537180435972196 ) ) ;
#28061=CARTESIAN_POINT ( 'NONE',  ( -11.25000000000000000, 12.50000000000000000, -7.122917578226813262 ) ) ;
#28062=CARTESIAN_POINT ( 'NONE',  ( 9.999999999999911182, 2.500000000000000000, 5.122947341949749323 ) ) ;
#28063=CARTESIAN_POINT ( 'NONE',  ( -5.650000000000019895, 2.500000000000000000, 1.918653347947321564 ) ) ;
#28064=VECTOR ( 'NONE', #66778, 1000.000000000000000 ) ;
#28065=ORIENTED_EDGE ( 'NONE', *, *, #41935, .F. ) ;
#28066=ORIENTED_EDGE ( 'NONE', *, *, #106160, .F. ) ;
#28067=ADVANCED_FACE ( 'NONE', ( #116595 ), #57025, .T. ) ;
#28068=VERTEX_POINT ( 'NONE', #34360 ) ;
#28069=DIRECTION ( 'NONE',  ( 0.000000000000000000, 0.000000000000000000, 1.000000000000000000 ) ) ;
#28070=DIRECTION ( 'NONE',  ( -4.274815082592931898E-19, -0.9999939076577903929, -0.003490651415223739937 ) ) ;
#28071=PLANE ( 'NONE',  #4112 ) ;
#28072=ORIENTED_EDGE ( 'NONE', *, *, #19260, .T. ) ;
#28073=ORIENTED_EDGE ( 'NONE', *, *, #74952, .F. ) ;
#28074=ORIENTED_EDGE ( 'NONE', *, *, #37097, .T. ) ;
#28075=FACE_OUTER_BOUND ( 'NONE', #92954, .T. ) ;
#28076=AXIS2_PLACEMENT_3D ( 'NONE', #109811, #106731, #59446 ) ;
#28077=LINE ( 'NONE', #7776, #92512 ) ;
#28079=DIRECTION ( 'NONE',  ( -0.000000000000000000, -1.000000000000000000, -0.000000000000000000 ) ) ;
#28080=DIRECTION ( 'NONE',  ( 0.000000000000000000, 1.000000000000000000, 0.000000000000000000 ) ) ;
#28081=CARTESIAN_POINT ( 'NONE',  ( 6.899999999999926636, 2.500000000000000000, -0.2464101615137782308 ) ) ;
#28082=CARTESIAN_POINT ( 'NONE',  ( -6.900000000000015454, 2.500000000000000000, 3.983716857408420076 ) ) ;
#28083=CARTESIAN_POINT ( 'NONE',  ( 0.6499999999999561684, 2.500000000000000000, 2.511473670974873507 ) ) ;
#28084=DIRECTION ( 'NONE',  ( 0.000000000000000000, -0.000000000000000000, 1.000000000000000000 ) ) ;
#28085=ORIENTED_EDGE ( 'NONE', *, *, #75489, .T. ) ;
#28086=ORIENTED_EDGE ( 'NONE', *, *, #39967, .F. ) ;
#28087=AXIS2_PLACEMENT_3D ( 'NONE', #68375, #78215, #18630 ) ;
#28088=DIRECTION ( 'NONE',  ( -4.274815082592931898E-19, -0.9999939076577903929, -0.003490651415223739937 ) ) ;
#28089=DIRECTION ( 'NONE',  ( 0.000000000000000000, 0.000000000000000000, -1.000000000000000000 ) ) ;
#28090=ORIENTED_EDGE ( 'NONE', *, *, #103481, .T. ) ;
#28091=ORIENTED_EDGE ( 'NONE', *, *, #2756, .F. ) ;
#28093=DIRECTION ( 'NONE',  ( 0.000000000000000000, 0.000000000000000000, -1.000000000000000000 ) ) ;
#28094=DIRECTION ( 'NONE',  ( 0.000000000000000000, -0.9999939076577903929, 0.003490651415223739937 ) ) ;
#28095=CARTESIAN_POINT ( 'NONE',  ( 11.24999999999994493, 2.500000000000000000, -2.165063509461101710 ) ) ;
#28097=VECTOR ( 'NONE', #91103, 1000.000000000000000 ) ;
#28098=FACE_OUTER_BOUND ( 'NONE', #113668, .T. ) ;
#28099=CIRCLE ( 'NONE', #49048, 0.06509327318403745899 ) ;
#28100=DIRECTION ( 'NONE',  ( 0.000000000000000000, 1.000000000000000000, 0.000000000000000000 ) ) ;
#28101=ORIENTED_EDGE ( 'NONE', *, *, #26705, .T. ) ;
#28102=DIRECTION ( 'NONE',  ( 0.000000000000000000, 0.000000000000000000, -1.000000000000000000 ) ) ;
#28104=CIRCLE ( 'NONE', #90791, 0.1000000000000000056 ) ;
#28105=CARTESIAN_POINT ( 'NONE',  ( 12.49999999999990230, 2.500000000000000000, -0.6928203230275541413 ) ) ;
#28106=EDGE_CURVE ( 'NONE', #117378, #111575, #125759, .T. ) ;
#28108=EDGE_LOOP ( 'NONE', ( #96840, #35753, #80213, #108616 ) ) ;
#28109=EDGE_CURVE ( 'NONE', #62965, #63975, #31796, .T. ) ;
#28110=ORIENTED_EDGE ( 'NONE', *, *, #31836, .T. ) ;
#28112=EDGE_CURVE ( 'NONE', #11241, #52697, #106980, .T. ) ;
#28113=CARTESIAN_POINT ( 'NONE',  ( -10.60000000000000142, 2.500000000000000000, 0.2464101615137736789 ) ) ;
#28114=CARTESIAN_POINT ( 'NONE',  ( 2.949999999999945111, 12.50000000000000000, 2.099970236277060032 ) ) ;
#28115=ORIENTED_EDGE ( 'NONE', *, *, #66266, .F. ) ;
#28116=DIRECTION ( 'NONE',  ( 0.000000000000000000, -0.000000000000000000, 1.000000000000000000 ) ) ;
#28117=CARTESIAN_POINT ( 'NONE',  ( 17.50000000000000000, 2.750000000000000000, -3.999999999999998224 ) ) ;
#28118=CIRCLE ( 'NONE', #46903, 0.1000000000000002554 ) ;
#28119=EDGE_CURVE ( 'NONE', #3070, #121018, #90253, .T. ) ;
#28120=CONICAL_SURFACE ( 'NONE', #78210, 0.1000000000000002554, 0.003490658503988666988 ) ;
#28121=FACE_OUTER_BOUND ( 'NONE', #22848, .T. ) ;
#28122=CARTESIAN_POINT ( 'NONE',  ( -10.65000000000000391, 12.50000000000000000, -2.576566944158911188 ) ) ;
#28123=ADVANCED_FACE ( 'NONE', ( #87136 ), #102779, .T. ) ;
#28124=ORIENTED_EDGE ( 'NONE', *, *, #33883, .T. ) ;
#28125=VECTOR ( 'NONE', #73634, 1000.000000000000000 ) ;
#28126=VECTOR ( 'NONE', #92773, 1000.000000000000000 ) ;
#28127=EDGE_CURVE ( 'NONE', #4240, #39644, #40106, .T. ) ;
#28128=CARTESIAN_POINT ( 'NONE',  ( -4.400000000000025224, 12.50000000000000000, 4.611443907251934426 ) ) ;
#28129=DIRECTION ( 'NONE',  ( 0.000000000000000000, 1.000000000000000000, 0.000000000000000000 ) ) ;
#28130=VERTEX_POINT ( 'NONE', #96959 ) ;
#28131=AXIS2_PLACEMENT_3D ( 'NONE', #89572, #69938, #109865 ) ;
#28132=AXIS2_PLACEMENT_3D ( 'NONE', #17051, #54432, #44625 ) ;
#28133=VECTOR ( 'NONE', #84635, 1000.000000000000000 ) ;
#28134=ORIENTED_EDGE ( 'NONE', *, *, #126215, .F. ) ;
#28135=ORIENTED_EDGE ( 'NONE', *, *, #67657, .T. ) ;
#28136=CARTESIAN_POINT ( 'NONE',  ( 9.599999999999914380, 12.50000000000000000, 4.330127018922196314 ) ) ;
#28137=DIRECTION ( 'NONE',  ( 0.000000000000000000, 0.000000000000000000, -1.000000000000000000 ) ) ;
#28138=CONICAL_SURFACE ( 'NONE', #101299, 0.1000000000000002554, 0.003490658503988666988 ) ;
#28139=AXIS2_PLACEMENT_3D ( 'NONE', #85005, #85655, #45103 ) ;
#28140=AXIS2_PLACEMENT_3D ( 'NONE', #96661, #120199, #39730 ) ;
#28141=EDGE_LOOP ( 'NONE', ( #98036, #88352, #41696, #37971 ) ) ;
#28142=CARTESIAN_POINT ( 'NONE',  ( -4.600000000000024514, 12.50000000000000000, 5.022947341949748790 ) ) ;
#28143=CARTESIAN_POINT ( 'NONE',  ( -1.250000000000037970, 2.500000000000000000, 7.188010851410848723 ) ) ;
#28144=DIRECTION ( 'NONE',  ( 0.000000000000000000, 0.000000000000000000, -1.000000000000000000 ) ) ;
#28145=DIRECTION ( 'NONE',  ( 0.000000000000000000, 1.000000000000000000, 0.000000000000000000 ) ) ;
#28146=EDGE_LOOP ( 'NONE', ( #4665, #26954 ) ) ;
#28147=PLANE ( 'NONE',  #43672 ) ;
#28148=ORIENTED_EDGE ( 'NONE', *, *, #50888, .F. ) ;
#28149=ORIENTED_EDGE ( 'NONE', *, *, #87530, .F. ) ;
#28150=DIRECTION ( 'NONE',  ( 0.000000000000000000, -0.000000000000000000, 1.000000000000000000 ) ) ;
#28151=CARTESIAN_POINT ( 'NONE',  ( 11.04999999999990656, 12.50000000000000000, 2.511473670974873507 ) ) ;
#28152=FACE_BOUND ( 'NONE', #91597, .T. ) ;
#28153=DIRECTION ( 'NONE',  ( 0.000000000000000000, 0.000000000000000000, 1.000000000000000000 ) ) ;
#28154=AXIS2_PLACEMENT_3D ( 'NONE', #6030, #5395, #4100 ) ;
#28155=CARTESIAN_POINT ( 'NONE',  ( -2.700000000000029932, 2.500000000000000000, -4.576537180435977348 ) ) ;
#28156=DIRECTION ( 'NONE',  ( 0.000000000000000000, 0.000000000000000000, 1.000000000000000000 ) ) ;
#28157=EDGE_CURVE ( 'NONE', #86941, #69063, #61021, .T. ) ;
#28158=ORIENTED_EDGE ( 'NONE', *, *, #104223, .T. ) ;
#28159=ADVANCED_FACE ( 'NONE', ( #43537 ), #26304, .T. ) ;
#28160=DIRECTION ( 'NONE',  ( 0.000000000000000000, 1.000000000000000000, 0.000000000000000000 ) ) ;
#28161=DIRECTION ( 'NONE',  ( 0.000000000000000000, 1.000000000000000000, 0.000000000000000000 ) ) ;
#28162=CARTESIAN_POINT ( 'NONE',  ( -14.54999999999998472, 12.50000000000000000, 2.165063509461101265 ) ) ;
#28163=ADVANCED_FACE ( 'NONE', ( #113543 ), #7929, .T. ) ;
#28164=DIRECTION ( 'NONE',  ( -0.000000000000000000, -1.000000000000000000, -0.000000000000000000 ) ) ;
#28165=ORIENTED_EDGE ( 'NONE', *, *, #126756, .T. ) ;
#28166=AXIS2_PLACEMENT_3D ( 'NONE', #126208, #56163, #97385 ) ;
#28168=DIRECTION ( 'NONE',  ( -0.000000000000000000, -1.000000000000000000, -0.000000000000000000 ) ) ;
#28169=EDGE_CURVE ( 'NONE', #60091, #121535, #65217, .T. ) ;
#28170=EDGE_LOOP ( 'NONE', ( #103371, #34330, #27230, #76634 ) ) ;
#28171=EDGE_LOOP ( 'NONE', ( #56334, #114784, #29958, #74155 ) ) ;
#28172=DIRECTION ( 'NONE',  ( 0.000000000000000000, -0.000000000000000000, 1.000000000000000000 ) ) ;
#28173=DIRECTION ( 'NONE',  ( -0.000000000000000000, -1.000000000000000000, -0.000000000000000000 ) ) ;
#28174=FACE_BOUND ( 'NONE', #22265, .T. ) ;
#28175=DIRECTION ( 'NONE',  ( 0.000000000000000000, 0.000000000000000000, -1.000000000000000000 ) ) ;
#28176=EDGE_CURVE ( 'NONE', #14119, #64139, #4560, .T. ) ;
#28177=CONICAL_SURFACE ( 'NONE', #19869, 0.1000000000000002554, 0.003490658503988666988 ) ;
#28178=EDGE_CURVE ( 'NONE', #120246, #98907, #123364, .T. ) ;
#28179=VERTEX_POINT ( 'NONE', #77323 ) ;
#28180=LINE ( 'NONE', #68088, #69573 ) ;
#28181=AXIS2_PLACEMENT_3D ( 'NONE', #118486, #28840, #89041 ) ;
#28182=ORIENTED_EDGE ( 'NONE', *, *, #109428, .T. ) ;
#28183=ORIENTED_EDGE ( 'NONE', *, *, #16280, .F. ) ;
#28184=DIRECTION ( 'NONE',  ( 0.000000000000000000, 0.000000000000000000, -1.000000000000000000 ) ) ;
#28186=EDGE_CURVE ( 'NONE', #14788, #11702, #17172, .T. ) ;
#28187=ORIENTED_EDGE ( 'NONE', *, *, #81972, .T. ) ;
#28189=DIRECTION ( 'NONE',  ( 0.000000000000000000, -0.9999939076577903929, 0.003490651415223739937 ) ) ;
#28190=AXIS2_PLACEMENT_3D ( 'NONE', #111211, #121049, #111886 ) ;
#28191=AXIS2_PLACEMENT_3D ( 'NONE', #50406, #83593, #72484 ) ;
#28192=CARTESIAN_POINT ( 'NONE',  ( 3.949999999999941558, 12.50000000000000000, -1.818653347947326138 ) ) ;
#28193=DIRECTION ( 'NONE',  ( 0.000000000000000000, -0.000000000000000000, 1.000000000000000000 ) ) ;
#28194=AXIS2_PLACEMENT_3D ( 'NONE', #123454, #125402, #84174 ) ;
#28195=EDGE_LOOP ( 'NONE', ( #38481, #77465 ) ) ;
#28196=CARTESIAN_POINT ( 'NONE',  ( -1.250000000000037970, 2.500000000000000000, 7.188010851410848723 ) ) ;
#28197=DIRECTION ( 'NONE',  ( -0.000000000000000000, 1.000000000000000000, -0.000000000000000000 ) ) ;
#28198=CARTESIAN_POINT ( 'NONE',  ( -10.45000000000000462, 2.500000000000000000, -6.395190528383298378 ) ) ;
#28199=DIRECTION ( 'NONE',  ( 0.000000000000000000, 0.000000000000000000, 1.000000000000000000 ) ) ;
#28200=VERTEX_POINT ( 'NONE', #63808 ) ;
#28201=CARTESIAN_POINT ( 'NONE',  ( 14.14999999999989200, 12.50000000000000000, -2.165063509461101710 ) ) ;
#28203=CARTESIAN_POINT ( 'NONE',  ( 17.46754094667558377, 1.506946019333248898, 5.249106724335526941 ) ) ;
#28204=EDGE_LOOP ( 'NONE', ( #18163, #19868 ) ) ;
#28205=PLANE ( 'NONE',  #107825 ) ;
#28206=LINE ( 'NONE', #119159, #51545 ) ;
#28207=DIRECTION ( 'NONE',  ( -0.000000000000000000, 1.000000000000000000, -0.000000000000000000 ) ) ;
#28208=CIRCLE ( 'NONE', #122310, 0.06509327318403745899 ) ;
#28209=DIRECTION ( 'NONE',  ( -0.000000000000000000, -1.000000000000000000, -0.000000000000000000 ) ) ;
#28211=AXIS2_PLACEMENT_3D ( 'NONE', #27935, #58056, #30542 ) ;
#28212=DIRECTION ( 'NONE',  ( 0.000000000000000000, 1.000000000000000000, 0.000000000000000000 ) ) ;
#28213=DIRECTION ( 'NONE',  ( -4.274815082592931898E-19, -0.9999939076577903929, -0.003490651415223739937 ) ) ;
#28214=DIRECTION ( 'NONE',  ( -4.274815082592931898E-19, -0.9999939076577903929, -0.003490651415223739937 ) ) ;
#28215=AXIS2_PLACEMENT_3D ( 'NONE', #113370, #103570, #72179 ) ;
#28216=DIRECTION ( 'NONE',  ( -0.000000000000000000, -1.000000000000000000, -0.000000000000000000 ) ) ;
#28217=CARTESIAN_POINT ( 'NONE',  ( -2.950000000000030376, 2.500000000000000000, 6.395190528383296602 ) ) ;
#28218=CARTESIAN_POINT ( 'NONE',  ( -4.350000000000023626, 2.500000000000000000, 2.411473670974873862 ) ) ;
#28219=VECTOR ( 'NONE', #31635, 1000.000000000000000 ) ;
#28220=ORIENTED_EDGE ( 'NONE', *, *, #70111, .T. ) ;
#28221=EDGE_CURVE ( 'NONE', #82798, #62529, #44157, .T. ) ;
#28222=CIRCLE ( 'NONE', #5217, 0.06509327318403745899 ) ;
#28223=VERTEX_POINT ( 'NONE', #106143 ) ;
#28224=CONICAL_SURFACE ( 'NONE', #101385, 0.1000000000000002554, 0.003490658503988666988 ) ;
#28225=CARTESIAN_POINT ( 'NONE',  ( 8.749999999999921840, 2.500000000000000000, 2.857883832488649301 ) ) ;
#28226=VERTEX_POINT ( 'NONE', #103736 ) ;
#28227=DIRECTION ( 'NONE',  ( 0.000000000000000000, 1.000000000000000000, 0.000000000000000000 ) ) ;
#28228=AXIS2_PLACEMENT_3D ( 'NONE', #23446, #63380, #115685 ) ;
#28229=VERTEX_POINT ( 'NONE', #67475 ) ;
#28230=ORIENTED_EDGE ( 'NONE', *, *, #38468, .F. ) ;
#28231=ORIENTED_EDGE ( 'NONE', *, *, #90789, .F. ) ;
#28232=DIRECTION ( 'NONE',  ( 0.000000000000000000, -0.000000000000000000, 1.000000000000000000 ) ) ;
#28233=LINE ( 'NONE', #30177, #52713 ) ;
#28234=CONICAL_SURFACE ( 'NONE', #26176, 0.1000000000000002554, 0.003490658503988666988 ) ;
#28235=CARTESIAN_POINT ( 'NONE',  ( -2.500000000000032419, 2.500000000000000000, 0.6928203230275494784 ) ) ;
#28236=DIRECTION ( 'NONE',  ( -0.000000000000000000, 1.000000000000000000, -0.000000000000000000 ) ) ;
#28237=DIRECTION ( 'NONE',  ( 0.000000000000000000, 0.000000000000000000, -1.000000000000000000 ) ) ;
#28238=VECTOR ( 'NONE', #55797, 1000.000000000000000 ) ;
#28239=CARTESIAN_POINT ( 'NONE',  ( -3.100000000000028955, 12.50000000000000000, 4.611443907251934426 ) ) ;
#28240=FACE_OUTER_BOUND ( 'NONE', #121858, .T. ) ;
#28241=DIRECTION ( 'NONE',  ( -0.000000000000000000, -1.000000000000000000, -0.000000000000000000 ) ) ;
#28242=ORIENTED_EDGE ( 'NONE', *, *, #71396, .T. ) ;
#28243=ORIENTED_EDGE ( 'NONE', *, *, #39421, .T. ) ;
#28244=VERTEX_POINT ( 'NONE', #17747 ) ;
#28245=DIRECTION ( 'NONE',  ( 0.000000000000000000, -0.9999939076577903929, 0.003490651415223739937 ) ) ;
#28246=ORIENTED_EDGE ( 'NONE', *, *, #86622, .F. ) ;
#28247=ORIENTED_EDGE ( 'NONE', *, *, #2173, .F. ) ;
#28248=AXIS2_PLACEMENT_3D ( 'NONE', #98363, #8683, #48637 ) ;
#28250=CARTESIAN_POINT ( 'NONE',  ( 8.749999999999920064, 2.500000000000000000, -2.857883832488653741 ) ) ;
#28251=DIRECTION ( 'NONE',  ( -0.000000000000000000, -1.000000000000000000, -0.000000000000000000 ) ) ;
#28252=DIRECTION ( 'NONE',  ( 0.000000000000000000, 1.000000000000000000, 0.000000000000000000 ) ) ;
#28253=DIRECTION ( 'NONE',  ( 0.000000000000000000, 0.000000000000000000, -1.000000000000000000 ) ) ;
#28254=ORIENTED_EDGE ( 'NONE', *, *, #63067, .F. ) ;
#28255=EDGE_CURVE ( 'NONE', #45160, #98077, #93913, .T. ) ;
#28256=DIRECTION ( 'NONE',  ( 0.000000000000000000, 1.000000000000000000, 0.000000000000000000 ) ) ;
#28257=AXIS2_PLACEMENT_3D ( 'NONE', #101128, #71663, #71028 ) ;
#28258=AXIS2_PLACEMENT_3D ( 'NONE', #48294, #100599, #88184 ) ;
#28259=VERTEX_POINT ( 'NONE', #53983 ) ;
#28260=DIRECTION ( 'NONE',  ( -0.000000000000000000, 1.000000000000000000, -0.000000000000000000 ) ) ;
#28261=ADVANCED_FACE ( 'NONE', ( #39364 ), #9877, .T. ) ;
#28262=EDGE_LOOP ( 'NONE', ( #21531, #60440 ) ) ;
#28263=CARTESIAN_POINT ( 'NONE',  ( -4.150000000000025224, 12.50000000000000000, -1.407149913249512663 ) ) ;
#28264=EDGE_LOOP ( 'NONE', ( #94205, #47057, #37085, #46226 ) ) ;
#28265=EDGE_CURVE ( 'NONE', #121714, #36406, #28233, .T. ) ;
#28266=ORIENTED_EDGE ( 'NONE', *, *, #125776, .F. ) ;
#28267=EDGE_CURVE ( 'NONE', #19758, #57799, #19246, .T. ) ;
#28268=DIRECTION ( 'NONE',  ( 0.000000000000000000, 1.000000000000000000, 0.000000000000000000 ) ) ;
#28269=CARTESIAN_POINT ( 'NONE',  ( 10.39999999999991154, 2.500000000000000000, 4.922947341949748257 ) ) ;
#28270=AXIS2_PLACEMENT_3D ( 'NONE', #112024, #24931, #121829 ) ;
#28271=DIRECTION ( 'NONE',  ( 0.000000000000000000, 1.000000000000000000, 0.000000000000000000 ) ) ;
#28272=CARTESIAN_POINT ( 'NONE',  ( 3.949999999999940670, 2.500000000000000000, 1.818653347947321475 ) ) ;
#28273=ADVANCED_FACE ( 'NONE', ( #28884 ), #2616, .T. ) ;
#28274=LINE ( 'NONE', #18448, #114093 ) ;
#28275=EDGE_CURVE ( 'NONE', #26422, #57522, #75779, .T. ) ;
#28276=ORIENTED_EDGE ( 'NONE', *, *, #11623, .T. ) ;
#28277=CARTESIAN_POINT ( 'NONE',  ( 3.949999999999938005, 2.500000000000000000, 6.941600689897073018 ) ) ;
#28278=DIRECTION ( 'NONE',  ( 0.000000000000000000, 0.000000000000000000, -1.000000000000000000 ) ) ;
#28279=EDGE_CURVE ( 'NONE', #51573, #12542, #73631, .T. ) ;
#28280=DIRECTION ( 'NONE',  ( -0.000000000000000000, 1.000000000000000000, -0.000000000000000000 ) ) ;
#28281=EDGE_CURVE ( 'NONE', #121393, #36999, #18405, .T. ) ;
#28282=ADVANCED_FACE ( 'NONE', ( #98245 ), #79905, .T. ) ;
#28283=CARTESIAN_POINT ( 'NONE',  ( -4.800000000000024691, 2.500000000000000000, 0.4464101615137735513 ) ) ;
#28284=CARTESIAN_POINT ( 'NONE',  ( 4.549999999999939426, 12.50000000000000000, -6.560283801567339701 ) ) ;
#28285=ORIENTED_EDGE ( 'NONE', *, *, #118703, .T. ) ;
#28286=CIRCLE ( 'NONE', #82677, 0.06509327318403745899 ) ;
#28287=CONICAL_SURFACE ( 'NONE', #30451, 0.09999999999999982514, 0.003490658503988666988 ) ;
#28288=VERTEX_POINT ( 'NONE', #99558 ) ;
#28289=DIRECTION ( 'NONE',  ( 0.000000000000000000, 0.000000000000000000, 1.000000000000000000 ) ) ;
#28291=ORIENTED_EDGE ( 'NONE', *, *, #77132, .F. ) ;
#28292=DIRECTION ( 'NONE',  ( 0.000000000000000000, 0.000000000000000000, 1.000000000000000000 ) ) ;
#28294=VERTEX_POINT ( 'NONE', #119185 ) ;
#28296=DIRECTION ( 'NONE',  ( -0.000000000000000000, -1.000000000000000000, -0.000000000000000000 ) ) ;
#28297=DIRECTION ( 'NONE',  ( -4.274815082592931898E-19, -0.9999939076577903929, -0.003490651415223739937 ) ) ;
#28298=AXIS2_PLACEMENT_3D ( 'NONE', #113888, #5839, #75884 ) ;
#28299=DIRECTION ( 'NONE',  ( 0.000000000000000000, 0.000000000000000000, 1.000000000000000000 ) ) ;
#28300=ORIENTED_EDGE ( 'NONE', *, *, #112280, .T. ) ;
#28301=CIRCLE ( 'NONE', #107718, 0.09999999999999999167 ) ;
#28302=CARTESIAN_POINT ( 'NONE',  ( 10.84999999999990905, 12.50000000000000000, 2.792790559304612064 ) ) ;
#28303=CONICAL_SURFACE ( 'NONE', #74279, 0.1000000000000002554, 0.003490658503988666988 ) ;
#28304=EDGE_LOOP ( 'NONE', ( #67637, #6082 ) ) ;
#28305=AXIS2_PLACEMENT_3D ( 'NONE', #86484, #127076, #104199 ) ;
#28306=DIRECTION ( 'NONE',  ( 0.000000000000000000, 0.000000000000000000, 1.000000000000000000 ) ) ;
#28307=CARTESIAN_POINT ( 'NONE',  ( -10.00000000000000355, 2.500000000000000000, 3.737306695894644371 ) ) ;
#28308=CARTESIAN_POINT ( 'NONE',  ( 8.549999999999922551, 12.50000000000000000, 2.511473670974873507 ) ) ;
#28309=AXIS2_PLACEMENT_3D ( 'NONE', #42769, #53216, #113407 ) ;
#28310=AXIS2_PLACEMENT_3D ( 'NONE', #39185, #107247, #58172 ) ;
#28311=ORIENTED_EDGE ( 'NONE', *, *, #3650, .T. ) ;
#28312=AXIS2_PLACEMENT_3D ( 'NONE', #5385, #95714, #103605 ) ;
#28313=CARTESIAN_POINT ( 'NONE',  ( -0.8500000000000382805, 2.500000000000000000, -2.957883832488653830 ) ) ;
#28314=CONICAL_SURFACE ( 'NONE', #24112, 0.1000000000000002554, 0.003490658503988666988 ) ;
#28315=ORIENTED_EDGE ( 'NONE', *, *, #69473, .F. ) ;
#28316=EDGE_CURVE ( 'NONE', #84188, #102542, #458, .T. ) ;
#28317=DIRECTION ( 'NONE',  ( -0.000000000000000000, -1.000000000000000000, -0.000000000000000000 ) ) ;
#28318=DIRECTION ( 'NONE',  ( -0.000000000000000000, 1.000000000000000000, -0.000000000000000000 ) ) ;
#28319=CARTESIAN_POINT ( 'NONE',  ( 12.69999999999990337, 2.500000000000000000, -4.676537180435978769 ) ) ;
#28320=ADVANCED_FACE ( 'NONE', ( #110019 ), #88288, .T. ) ;
#28321=ORIENTED_EDGE ( 'NONE', *, *, #8365, .F. ) ;
#28322=AXIS2_PLACEMENT_3D ( 'NONE', #103120, #123396, #4902 ) ;
#28323=DIRECTION ( 'NONE',  ( 0.000000000000000000, -0.9999939076577903929, 0.003490651415223739937 ) ) ;
#28324=EDGE_CURVE ( 'NONE', #70717, #53411, #11150, .T. ) ;
#28325=CIRCLE ( 'NONE', #17846, 0.06509327318403745899 ) ;
#28326=CARTESIAN_POINT ( 'NONE',  ( -4.150000000000025224, 2.500000000000000000, 6.495190528383297135 ) ) ;
#28327=CIRCLE ( 'NONE', #45063, 0.06509327318403745899 ) ;
#28328=ORIENTED_EDGE ( 'NONE', *, *, #18913, .F. ) ;
#28329=DIRECTION ( 'NONE',  ( 0.000000000000000000, 0.000000000000000000, 1.000000000000000000 ) ) ;
#28330=EDGE_CURVE ( 'NONE', #58403, #37993, #68793, .T. ) ;
#28331=EDGE_LOOP ( 'NONE', ( #27422, #96551, #90662, #28496 ) ) ;
#28332=DIRECTION ( 'NONE',  ( 0.000000000000000000, 0.000000000000000000, 1.000000000000000000 ) ) ;
#28333=ADVANCED_FACE ( 'NONE', ( #58980 ), #94562, .T. ) ;
#28334=EDGE_CURVE ( 'NONE', #92046, #126222, #86137, .T. ) ;
#28335=ADVANCED_FACE ( 'NONE', ( #89720 ), #90349, .T. ) ;
#28336=ORIENTED_EDGE ( 'NONE', *, *, #64731, .F. ) ;
#28337=FACE_OUTER_BOUND ( 'NONE', #3699, .T. ) ;
#28338=CARTESIAN_POINT ( 'NONE',  ( -2.900000000000029221, 12.50000000000000000, -0.6928203230275541413 ) ) ;
#28339=VERTEX_POINT ( 'NONE', #46 ) ;
#28340=ORIENTED_EDGE ( 'NONE', *, *, #24868, .T. ) ;
#28341=CARTESIAN_POINT ( 'NONE',  ( -5.450000000000023270, 2.500000000000000000, -2.265063509461101798 ) ) ;
#28343=CIRCLE ( 'NONE', #114024, 0.06509327318403745899 ) ;
#28344=VERTEX_POINT ( 'NONE', #40654 ) ;
#28345=ADVANCED_FACE ( 'NONE', ( #80559 ), #110648, .T. ) ;
#28348=DIRECTION ( 'NONE',  ( 0.000000000000000000, 0.000000000000000000, -1.000000000000000000 ) ) ;
#28349=DIRECTION ( 'NONE',  ( 0.000000000000000000, 1.000000000000000000, 0.000000000000000000 ) ) ;
#28350=DIRECTION ( 'NONE',  ( 0.000000000000000000, 0.000000000000000000, -1.000000000000000000 ) ) ;
#28351=CIRCLE ( 'NONE', #95251, 0.06509327318403745899 ) ;
#28352=DIRECTION ( 'NONE',  ( -0.000000000000000000, 1.000000000000000000, -0.000000000000000000 ) ) ;
#28353=AXIS2_PLACEMENT_3D ( 'NONE', #102398, #52636, #92570 ) ;
#28354=CIRCLE ( 'NONE', #11616, 0.1000000000000002554 ) ;
#28355=VERTEX_POINT ( 'NONE', #111267 ) ;
#28356=EDGE_LOOP ( 'NONE', ( #35725, #111168, #91710, #86549 ) ) ;
#28357=ORIENTED_EDGE ( 'NONE', *, *, #94927, .F. ) ;
#28358=ORIENTED_EDGE ( 'NONE', *, *, #66384, .F. ) ;
#28359=DIRECTION ( 'NONE',  ( 0.000000000000000000, 0.000000000000000000, 1.000000000000000000 ) ) ;
#28361=FACE_OUTER_BOUND ( 'NONE', #48251, .T. ) ;
#28362=ORIENTED_EDGE ( 'NONE', *, *, #79261, .T. ) ;
#28363=FACE_BOUND ( 'NONE', #95157, .T. ) ;
#28364=ORIENTED_EDGE ( 'NONE', *, *, #28852, .T. ) ;
#28365=EDGE_CURVE ( 'NONE', #72890, #53599, #19341, .T. ) ;
#28366=DIRECTION ( 'NONE',  ( 0.000000000000000000, 0.000000000000000000, -1.000000000000000000 ) ) ;
#28367=LINE ( 'NONE', #116724, #110735 ) ;
#28368=AXIS2_PLACEMENT_3D ( 'NONE', #48433, #110577, #69350 ) ;
#28369=DIRECTION ( 'NONE',  ( 0.000000000000000000, 1.000000000000000000, 0.000000000000000000 ) ) ;
#28370=DIRECTION ( 'NONE',  ( 0.000000000000000000, 0.000000000000000000, -1.000000000000000000 ) ) ;
#28371=CIRCLE ( 'NONE', #107778, 0.09999999999999999167 ) ;
#28372=CARTESIAN_POINT ( 'NONE',  ( 10.64999999999991331, 2.500000000000000000, -2.511473670974877948 ) ) ;
#28373=FACE_OUTER_BOUND ( 'NONE', #16661, .T. ) ;
#28374=DIRECTION ( 'NONE',  ( 0.000000000000000000, 1.000000000000000000, 0.000000000000000000 ) ) ;
#28375=DIRECTION ( 'NONE',  ( -0.000000000000000000, 1.000000000000000000, -0.000000000000000000 ) ) ;
#28376=DIRECTION ( 'NONE',  ( 0.000000000000000000, 0.000000000000000000, 1.000000000000000000 ) ) ;
#28377=DIRECTION ( 'NONE',  ( 0.000000000000000000, 1.000000000000000000, 0.000000000000000000 ) ) ;
#28378=AXIS2_PLACEMENT_3D ( 'NONE', #68898, #10601, #128495 ) ;
#28379=EDGE_LOOP ( 'NONE', ( #76009, #105372, #64495, #86529 ) ) ;
#28380=ORIENTED_EDGE ( 'NONE', *, *, #118599, .T. ) ;
#28381=CIRCLE ( 'NONE', #53515, 0.1000000000000002554 ) ;
#28382=ADVANCED_FACE ( 'NONE', ( #2612 ), #72670, .T. ) ;
#28383=ORIENTED_EDGE ( 'NONE', *, *, #29904, .T. ) ;
#28384=ORIENTED_EDGE ( 'NONE', *, *, #27785, .T. ) ;
#28385=CARTESIAN_POINT ( 'NONE',  ( 17.50000000000010303, -2.262036863574762080, -3.993716676846037039 ) ) ;
#28386=FACE_OUTER_BOUND ( 'NONE', #31820, .T. ) ;
#28387=ORIENTED_EDGE ( 'NONE', *, *, #122864, .T. ) ;
#28388=EDGE_LOOP ( 'NONE', ( #8754, #14308, #75389, #77275 ) ) ;
#28389=ORIENTED_EDGE ( 'NONE', *, *, #13815, .F. ) ;
#28390=DIRECTION ( 'NONE',  ( 0.000000000000000000, 1.000000000000000000, 0.000000000000000000 ) ) ;
#28391=LINE ( 'NONE', #68295, #69714 ) ;
#28393=CARTESIAN_POINT ( 'NONE',  ( 5.399999999999932854, 12.50000000000000000, 5.022947341949748790 ) ) ;
#28394=CARTESIAN_POINT ( 'NONE',  ( -13.54999999999999005, 2.500000000000000000, 2.411473670974877415 ) ) ;
#28395=PLANE ( 'NONE',  #37216 ) ;
#28396=PLANE ( 'NONE',  #44493 ) ;
#28397=EDGE_CURVE ( 'NONE', #2959, #41590, #100815, .T. ) ;
#28398=ORIENTED_EDGE ( 'NONE', *, *, #61896, .F. ) ;
#28399=LINE ( 'NONE', #9402, #39252 ) ;
#28400=VERTEX_POINT ( 'NONE', #73295 ) ;
#28401=AXIS2_PLACEMENT_3D ( 'NONE', #80046, #20491, #70232 ) ;
#28402=VERTEX_POINT ( 'NONE', #64125 ) ;
#28403=VERTEX_POINT ( 'NONE', #14365 ) ;
#28404=AXIS2_PLACEMENT_3D ( 'NONE', #36176, #13934, #65616 ) ;
#28405=CARTESIAN_POINT ( 'NONE',  ( -10.00000000000000533, 12.50000000000000000, 0.7579135962115869374 ) ) ;
#28406=( BOUNDED_SURFACE ( )  B_SPLINE_SURFACE ( 3, 2, ( 
 ( #51022, #1894, #77089 ),
 ( #116354, #56144, #84325 ),
 ( #94146, #37177, #126185 ),
 ( #16838, #24127, #5743 ),
 ( #36537, #45705, #105904 ),
 ( #16207, #75158, #96078 ),
 ( #44405, #6375, #46330 ),
 ( #86242, #125534, #65317 ),
 ( #76447, #115055, #26058 ),
 ( #45068, #105254, #5111 ),
 ( #64046, #24773, #85612 ),
 ( #94794, #115709, #64683 ),
 ( #4444, #35877, #15573 ),
 ( #26698, #25389, #55521 ) ),
 .UNSPECIFIED., .F., .F., .F. ) 
 B_SPLINE_SURFACE_WITH_KNOTS ( ( 4, 2, 2, 2, 2, 2, 4 ),
 ( 3, 3 ),
 ( 0.000000000000000000, 0.001744612550434199941, 0.002616918825651300129, 0.003489225100868399883, 0.005233837651302600258, 0.006106143926519700012, 0.006978450201736799766 ),
 ( 0.000000000000000000, 1.000000000000000000 ),
 .UNSPECIFIED. ) 
 GEOMETRIC_REPRESENTATION_ITEM ( )  RATIONAL_B_SPLINE_SURFACE ( (
 ( 1.000000000000000000, 0.7318752858502181047, 1.000000000000000000),
 ( 1.000000000000000000, 0.7270130115578827823, 1.000000000000000000),
 ( 1.000000000000000000, 0.7223762446139352367, 1.000000000000000000),
 ( 1.000000000000000000, 0.7156127915551185881, 1.000000000000000000),
 ( 1.000000000000000000, 0.7133893117692130525, 1.000000000000000000),
 ( 1.000000000000000000, 0.7090389252573708889, 1.000000000000000000),
 ( 1.000000000000000000, 0.7069297463491673872, 1.000000000000000000),
 ( 1.000000000000000000, 0.7010696893200437652, 1.000000000000000000),
 ( 1.000000000000000000, 0.6977361265600255935, 1.000000000000000000),
 ( 1.000000000000000000, 0.6948030504687735531, 1.000000000000000000),
 ( 1.000000000000000000, 0.6942033558614377764, 1.000000000000000000),
 ( 1.000000000000000000, 0.6937817651809667918, 1.000000000000000000),
 ( 1.000000000000000000, 0.6939284133496244067, 1.000000000000000000),
 ( 1.000000000000000000, 0.6944177883068211043, 1.000000000000000000) ) ) 
 REPRESENTATION_ITEM ( '' )  SURFACE ( )  );
#28407=ORIENTED_EDGE ( 'NONE', *, *, #87397, .F. ) ;
#28408=EDGE_LOOP ( 'NONE', ( #50937, #3857, #22322, #39492 ) ) ;
#28409=DIRECTION ( 'NONE',  ( 0.000000000000000000, 0.000000000000000000, 1.000000000000000000 ) ) ;
#28410=CARTESIAN_POINT ( 'NONE',  ( -14.54999999999998472, 2.500000000000000000, 2.165063509461101265 ) ) ;
#28411=FACE_OUTER_BOUND ( 'NONE', #128065, .T. ) ;
#28412=LINE ( 'NONE', #79450, #117325 ) ;
#28413=AXIS2_PLACEMENT_3D ( 'NONE', #76268, #106365, #27797 ) ;
#28414=DIRECTION ( 'NONE',  ( 0.000000000000000000, 0.000000000000000000, 1.000000000000000000 ) ) ;
#28415=ORIENTED_EDGE ( 'NONE', *, *, #111934, .T. ) ;
#28416=CARTESIAN_POINT ( 'NONE',  ( -8.150000000000012790, 2.500000000000000000, -2.511473670974877948 ) ) ;
#28417=CIRCLE ( 'NONE', #68101, 0.1000000000000002554 ) ;
#28418=VECTOR ( 'NONE', #12416, 1000.000000000000000 ) ;
#28419=VERTEX_POINT ( 'NONE', #73951 ) ;
#28420=CARTESIAN_POINT ( 'NONE',  ( -3.100000000000028955, 12.50000000000000000, 3.983716857408420964 ) ) ;
#28421=CIRCLE ( 'NONE', #86988, 0.06509327318403745899 ) ;
#28423=VERTEX_POINT ( 'NONE', #71354 ) ;
#28425=DIRECTION ( 'NONE',  ( 0.000000000000000000, -0.000000000000000000, 1.000000000000000000 ) ) ;
#28426=AXIS2_PLACEMENT_3D ( 'NONE', #62104, #575, #42466 ) ;
#28427=ORIENTED_EDGE ( 'NONE', *, *, #29444, .F. ) ;
#28428=CARTESIAN_POINT ( 'NONE',  ( -10.20000000000000284, 2.500000000000000000, 3.983716857408420964 ) ) ;
#28429=DIRECTION ( 'NONE',  ( -0.000000000000000000, 1.000000000000000000, -0.000000000000000000 ) ) ;
#28430=EDGE_LOOP ( 'NONE', ( #17466, #63927, #121957, #113228 ) ) ;
#28431=CARTESIAN_POINT ( 'NONE',  ( 1.649999999999951505, 12.50000000000000000, -1.472243186433550122 ) ) ;
#28432=ORIENTED_EDGE ( 'NONE', *, *, #41924, .T. ) ;
#28433=EDGE_CURVE ( 'NONE', #104247, #113011, #63181, .T. ) ;
#28434=EDGE_CURVE ( 'NONE', #45891, #41822, #128023, .T. ) ;
#28435=ORIENTED_EDGE ( 'NONE', *, *, #62279, .T. ) ;
#28436=CARTESIAN_POINT ( 'NONE',  ( -6.850000000000017408, 12.50000000000000000, -1.883746621131363375 ) ) ;
#28437=DIRECTION ( 'NONE',  ( 0.000000000000000000, 1.000000000000000000, 0.000000000000000000 ) ) ;
#28438=EDGE_CURVE ( 'NONE', #117751, #50154, #46444, .T. ) ;
#28440=EDGE_CURVE ( 'NONE', #122530, #23542, #96605, .T. ) ;
#28441=CIRCLE ( 'NONE', #128806, 0.06509327318403745899 ) ;
#28442=CARTESIAN_POINT ( 'NONE',  ( 2.699999999999946443, 12.50000000000000000, -3.983716857408426293 ) ) ;
#28443=DIRECTION ( 'NONE',  ( 0.000000000000000000, -0.000000000000000000, 1.000000000000000000 ) ) ;
#28444=EDGE_CURVE ( 'NONE', #110699, #55428, #103416, .T. ) ;
#28447=ADVANCED_FACE ( 'NONE', ( #92959 ), #81202, .T. ) ;
#28448=ORIENTED_EDGE ( 'NONE', *, *, #30231, .T. ) ;
#28449=CIRCLE ( 'NONE', #84869, 0.06509327318403745899 ) ;
#28450=ADVANCED_FACE ( 'NONE', ( #61572 ), #3278, .T. ) ;
#28451=CARTESIAN_POINT ( 'NONE',  ( 9.799999999999913669, 12.50000000000000000, -3.983716857408426293 ) ) ;
#28452=CARTESIAN_POINT ( 'NONE',  ( -11.64999999999999680, 12.50000000000000000, 2.792790559304612064 ) ) ;
#28453=ADVANCED_FACE ( 'NONE', ( #53664 ), #31881, .T. ) ;
#28454=AXIS2_PLACEMENT_3D ( 'NONE', #105450, #75328, #115897 ) ;
#28455=ORIENTED_EDGE ( 'NONE', *, *, #4711, .T. ) ;
#28457=FACE_OUTER_BOUND ( 'NONE', #112395, .T. ) ;
#28458=CARTESIAN_POINT ( 'NONE',  ( 13.14999999999990088, 2.500000000000000000, 1.818653347947321475 ) ) ;
#28459=DIRECTION ( 'NONE',  ( -4.274815082592931898E-19, -0.9999939076577903929, -0.003490651415223739937 ) ) ;
#28461=EDGE_CURVE ( 'NONE', #116195, #111299, #75682, .T. ) ;
#28462=DIRECTION ( 'NONE',  ( 0.000000000000000000, 1.000000000000000000, 0.000000000000000000 ) ) ;
#28463=ORIENTED_EDGE ( 'NONE', *, *, #22204, .F. ) ;
#28464=CIRCLE ( 'NONE', #101625, 0.09999999999999982514 ) ;
#28465=CIRCLE ( 'NONE', #66009, 0.06509327318403741736 ) ;
#28466=DIRECTION ( 'NONE',  ( 0.000000000000000000, 0.000000000000000000, 1.000000000000000000 ) ) ;
#28467=DIRECTION ( 'NONE',  ( 0.000000000000000000, 1.000000000000000000, 0.000000000000000000 ) ) ;
#28468=ORIENTED_EDGE ( 'NONE', *, *, #101012, .T. ) ;
#28469=CARTESIAN_POINT ( 'NONE',  ( -1.450000000000035039, 2.500000000000000000, -2.411473670974877859 ) ) ;
#28470=VERTEX_POINT ( 'NONE', #24209 ) ;
#28471=VERTEX_POINT ( 'NONE', #104055 ) ;
#28473=ORIENTED_EDGE ( 'NONE', *, *, #95656, .F. ) ;
#28474=PLANE ( 'NONE',  #579 ) ;
#28476=DIRECTION ( 'NONE',  ( -0.000000000000000000, -1.000000000000000000, -0.000000000000000000 ) ) ;
#28477=EDGE_LOOP ( 'NONE', ( #51552, #74574, #53341, #52571 ) ) ;
#28478=DIRECTION ( 'NONE',  ( 0.000000000000000000, -0.000000000000000000, 1.000000000000000000 ) ) ;
#28479=LINE ( 'NONE', #40228, #22286 ) ;
#28480=ORIENTED_EDGE ( 'NONE', *, *, #110617, .T. ) ;
#28481=CARTESIAN_POINT ( 'NONE',  ( 12.89999999999990266, 2.500000000000000000, -3.637306695894650055 ) ) ;
#28482=DIRECTION ( 'NONE',  ( 0.000000000000000000, 0.000000000000000000, -1.000000000000000000 ) ) ;
#28483=EDGE_LOOP ( 'NONE', ( #113187, #52915 ) ) ;
#28484=ADVANCED_FACE ( 'NONE', ( #11801 ), #51741, .T. ) ;
#28485=ORIENTED_EDGE ( 'NONE', *, *, #639, .F. ) ;
#28486=AXIS2_PLACEMENT_3D ( 'NONE', #72082, #120527, #70775 ) ;
#28487=EDGE_CURVE ( 'NONE', #19960, #106590, #121750, .T. ) ;
#28488=ORIENTED_EDGE ( 'NONE', *, *, #25963, .T. ) ;
#28489=PLANE ( 'NONE',  #58846 ) ;
#28490=CARTESIAN_POINT ( 'NONE',  ( 11.24999999999990941, 12.50000000000000000, -1.407149913249512663 ) ) ;
#28491=FACE_OUTER_BOUND ( 'NONE', #5178, .T. ) ;
#28492=FACE_BOUND ( 'NONE', #28895, .T. ) ;
#28493=ORIENTED_EDGE ( 'NONE', *, *, #110889, .F. ) ;
#28495=CARTESIAN_POINT ( 'NONE',  ( 2.099999999999949463, 12.50000000000000000, -3.637306695894650055 ) ) ;
#28496=ORIENTED_EDGE ( 'NONE', *, *, #67725, .T. ) ;
#28497=EDGE_CURVE ( 'NONE', #71388, #35640, #8873, .T. ) ;
#28498=AXIS2_PLACEMENT_3D ( 'NONE', #44879, #75593, #53402 ) ;
#28499=AXIS2_PLACEMENT_3D ( 'NONE', #11587, #51528, #101907 ) ;
#28500=DIRECTION ( 'NONE',  ( 0.000000000000000000, 0.000000000000000000, -1.000000000000000000 ) ) ;
#28501=CARTESIAN_POINT ( 'NONE',  ( -9.400000000000009237, 12.50000000000000000, -4.676537180435974328 ) ) ;
#28502=DIRECTION ( 'NONE',  ( 0.000000000000000000, -0.9999939076577903929, 0.003490651415223739937 ) ) ;
#28503=CARTESIAN_POINT ( 'NONE',  ( -10.00000000000000711, 2.500000000000000000, -3.637306695894645614 ) ) ;
#28504=CARTESIAN_POINT ( 'NONE',  ( 17.50000000000000000, 2.500000000000000000, -2.922290670089280340 ) ) ;
#28505=DIRECTION ( 'NONE',  ( 0.000000000000000000, 0.000000000000000000, 1.000000000000000000 ) ) ;
#28506=DIRECTION ( 'NONE',  ( 0.000000000000000000, 0.000000000000000000, 1.000000000000000000 ) ) ;
#28507=AXIS2_PLACEMENT_3D ( 'NONE', #72867, #121969, #112796 ) ;
#28509=CIRCLE ( 'NONE', #87071, 0.06509327318403745899 ) ;
#28510=ORIENTED_EDGE ( 'NONE', *, *, #91218, .F. ) ;
#28511=ORIENTED_EDGE ( 'NONE', *, *, #29904, .F. ) ;
#28512=ORIENTED_EDGE ( 'NONE', *, *, #32433, .F. ) ;
#28513=VERTEX_POINT ( 'NONE', #25477 ) ;
#28514=ORIENTED_EDGE ( 'NONE', *, *, #36333, .T. ) ;
#28515=DIRECTION ( 'NONE',  ( -0.000000000000000000, 1.000000000000000000, -0.000000000000000000 ) ) ;
#28516=CARTESIAN_POINT ( 'NONE',  ( 11.24999999999994493, 2.500000000000000000, -2.165063509461101710 ) ) ;
#28517=EDGE_LOOP ( 'NONE', ( #106353, #107598, #43677, #31607 ) ) ;
#28518=FACE_BOUND ( 'NONE', #33640, .T. ) ;
#28519=DIRECTION ( 'NONE',  ( -0.000000000000000000, 1.000000000000000000, -0.000000000000000000 ) ) ;
#28520=DIRECTION ( 'NONE',  ( 0.000000000000000000, 0.000000000000000000, 1.000000000000000000 ) ) ;
#28521=CARTESIAN_POINT ( 'NONE',  ( 2.299999999999949640, 12.50000000000000000, -4.676537180435977881 ) ) ;
#28522=CARTESIAN_POINT ( 'NONE',  ( -6.850000000000017408, 2.500000000000000000, -1.818653347947325916 ) ) ;
#28523=DIRECTION ( 'NONE',  ( 0.000000000000000000, 0.000000000000000000, 1.000000000000000000 ) ) ;
#28524=CIRCLE ( 'NONE', #43293, 0.1000000000000002554 ) ;
#28525=VERTEX_POINT ( 'NONE', #46410 ) ;
#28526=CARTESIAN_POINT ( 'NONE',  ( 12.69999999999989804, 12.50000000000000000, 0.3464101615137735735 ) ) ;
#28527=ORIENTED_EDGE ( 'NONE', *, *, #80300, .T. ) ;
#28528=CONICAL_SURFACE ( 'NONE', #95425, 0.09999999999999982514, 0.003490658503988666988 ) ;
#28529=EDGE_LOOP ( 'NONE', ( #34449, #66550 ) ) ;
#28530=ORIENTED_EDGE ( 'NONE', *, *, #3846, .F. ) ;
#28531=DIRECTION ( 'NONE',  ( 0.000000000000000000, 1.000000000000000000, 0.000000000000000000 ) ) ;
#28532=CARTESIAN_POINT ( 'NONE',  ( 3.549999999999944755, 12.50000000000000000, -2.446380397790840266 ) ) ;
#28533=CARTESIAN_POINT ( 'NONE',  ( -5.200000000000020606, 12.50000000000000000, -0.3464101615137782364 ) ) ;
#28534=ORIENTED_EDGE ( 'NONE', *, *, #16883, .F. ) ;
#28535=DIRECTION ( 'NONE',  ( 0.000000000000000000, 1.000000000000000000, 0.000000000000000000 ) ) ;
#28536=AXIS2_PLACEMENT_3D ( 'NONE', #108511, #64238, #78439 ) ;
#28537=AXIS2_PLACEMENT_3D ( 'NONE', #62952, #120588, #72781 ) ;
#28538=DIRECTION ( 'NONE',  ( 0.000000000000000000, 0.000000000000000000, 1.000000000000000000 ) ) ;
#28539=VECTOR ( 'NONE', #32710, 1000.000000000000000 ) ;
#28540=DIRECTION ( 'NONE',  ( 0.000000000000000000, -0.000000000000000000, 1.000000000000000000 ) ) ;
#28542=DIRECTION ( 'NONE',  ( 0.000000000000000000, -0.000000000000000000, 1.000000000000000000 ) ) ;
#28543=CARTESIAN_POINT ( 'NONE',  ( 6.649999999999928413, 12.50000000000000000, 2.857883832488649301 ) ) ;
#28544=ADVANCED_FACE ( 'NONE', ( #17591 ), #126926, .T. ) ;
#28545=DIRECTION ( 'NONE',  ( 0.000000000000000000, 1.000000000000000000, 0.000000000000000000 ) ) ;
#28546=ADVANCED_FACE ( 'NONE', ( #67315 ), #115477, .T. ) ;
#28547=ORIENTED_EDGE ( 'NONE', *, *, #17766, .T. ) ;
#28548=CARTESIAN_POINT ( 'NONE',  ( -5.450000000000023270, 2.500000000000000000, -2.065063509461102065 ) ) ;
#28549=AXIS2_PLACEMENT_3D ( 'NONE', #35576, #74206, #44751 ) ;
#28550=ORIENTED_EDGE ( 'NONE', *, *, #114001, .F. ) ;
#28551=AXIS2_PLACEMENT_3D ( 'NONE', #111787, #122898, #43710 ) ;
#28552=AXIS2_PLACEMENT_3D ( 'NONE', #123197, #33530, #93727 ) ;
#28553=ORIENTED_EDGE ( 'NONE', *, *, #79641, .T. ) ;
#28554=DIRECTION ( 'NONE',  ( 0.000000000000000000, 1.000000000000000000, 0.000000000000000000 ) ) ;
#28555=DIRECTION ( 'NONE',  ( 0.000000000000000000, 0.000000000000000000, 1.000000000000000000 ) ) ;
#28556=CARTESIAN_POINT ( 'NONE',  ( 8.749999999999923617, 12.50000000000000000, -7.253104124594891289 ) ) ;
#28557=EDGE_CURVE ( 'NONE', #10201, #114690, #77841, .T. ) ;
#28558=ORIENTED_EDGE ( 'NONE', *, *, #6333, .T. ) ;
#28559=ORIENTED_EDGE ( 'NONE', *, *, #10121, .T. ) ;
#28560=DIRECTION ( 'NONE',  ( -0.000000000000000000, 1.000000000000000000, -0.000000000000000000 ) ) ;
#28561=DIRECTION ( 'NONE',  ( 0.000000000000000000, 1.000000000000000000, 0.000000000000000000 ) ) ;
#28562=DIRECTION ( 'NONE',  ( -0.000000000000000000, 1.000000000000000000, -0.000000000000000000 ) ) ;
#28563=ORIENTED_EDGE ( 'NONE', *, *, #110020, .T. ) ;
#28564=ORIENTED_EDGE ( 'NONE', *, *, #58484, .T. ) ;
#28565=CARTESIAN_POINT ( 'NONE',  ( 8.349999999999923261, 12.50000000000000000, 2.165063509461097713 ) ) ;
#28566=VERTEX_POINT ( 'NONE', #15652 ) ;
#28567=DIRECTION ( 'NONE',  ( 0.000000000000000000, 0.000000000000000000, -1.000000000000000000 ) ) ;
#28568=FACE_OUTER_BOUND ( 'NONE', #106617, .T. ) ;
#28569=ORIENTED_EDGE ( 'NONE', *, *, #15008, .F. ) ;
#28570=CARTESIAN_POINT ( 'NONE',  ( -7.700000000000016165, 2.500000000000000000, -3.983716857408426293 ) ) ;
#28571=ADVANCED_FACE ( 'NONE', ( #74594 ), #12986, .T. ) ;
#28572=CARTESIAN_POINT ( 'NONE',  ( 8.149999999999923972, 12.50000000000000000, -6.841600689897077814 ) ) ;
#28574=CARTESIAN_POINT ( 'NONE',  ( 6.899999999999928413, 12.50000000000000000, -3.983716857408426293 ) ) ;
#28575=ORIENTED_EDGE ( 'NONE', *, *, #68195, .F. ) ;
#28576=EDGE_CURVE ( 'NONE', #115529, #68346, #82045, .T. ) ;
#28577=DIRECTION ( 'NONE',  ( 0.000000000000000000, 0.000000000000000000, -1.000000000000000000 ) ) ;
#28578=AXIS2_PLACEMENT_3D ( 'NONE', #91000, #121736, #69413 ) ;
#28579=VECTOR ( 'NONE', #15702, 1000.000000000000000 ) ;
#28580=ORIENTED_EDGE ( 'NONE', *, *, #46969, .F. ) ;
#28581=ORIENTED_EDGE ( 'NONE', *, *, #108528, .T. ) ;
#28582=EDGE_CURVE ( 'NONE', #109502, #96511, #107082, .T. ) ;
#28583=EDGE_CURVE ( 'NONE', #21308, #92121, #76534, .T. ) ;
#28584=DIRECTION ( 'NONE',  ( 0.000000000000000000, 0.000000000000000000, 1.000000000000000000 ) ) ;
#28586=DIRECTION ( 'NONE',  ( 0.000000000000000000, 0.000000000000000000, 1.000000000000000000 ) ) ;
#28587=EDGE_CURVE ( 'NONE', #13480, #115977, #8880, .T. ) ;
#28588=LINE ( 'NONE', #86851, #114852 ) ;
#28590=DIRECTION ( 'NONE',  ( 0.000000000000000000, 0.000000000000000000, 1.000000000000000000 ) ) ;
#28591=AXIS2_PLACEMENT_3D ( 'NONE', #93019, #54368, #23622 ) ;
#28592=FACE_OUTER_BOUND ( 'NONE', #111102, .T. ) ;
#28593=CONICAL_SURFACE ( 'NONE', #70347, 0.09999999999999982514, 0.003490658503988666988 ) ;
#28594=DIRECTION ( 'NONE',  ( 0.000000000000000000, -0.000000000000000000, -1.000000000000000000 ) ) ;
#28595=DIRECTION ( 'NONE',  ( 0.000000000000000000, 0.000000000000000000, -1.000000000000000000 ) ) ;
#28596=LINE ( 'NONE', #48228, #127923 ) ;
#28597=EDGE_CURVE ( 'NONE', #79180, #103166, #113348, .T. ) ;
#28598=EDGE_CURVE ( 'NONE', #19791, #76524, #14997, .T. ) ;
#28599=CARTESIAN_POINT ( 'NONE',  ( -15.59999999999998010, 2.500000000000000000, 0.3464101615137759604 ) ) ;
#28600=VECTOR ( 'NONE', #733, 1000.000000000000000 ) ;
#28601=AXIS2_PLACEMENT_3D ( 'NONE', #18336, #109297, #19642 ) ;
#28602=EDGE_CURVE ( 'NONE', #17818, #100677, #33944, .T. ) ;
#28603=VECTOR ( 'NONE', #43496, 1000.000000000000000 ) ;
#28604=ADVANCED_FACE ( 'NONE', ( #116438 ), #50661, .T. ) ;
#28605=VERTEX_POINT ( 'NONE', #37261 ) ;
#28606=FACE_OUTER_BOUND ( 'NONE', #100642, .T. ) ;
#28607=EDGE_CURVE ( 'NONE', #59496, #65382, #98770, .T. ) ;
#28608=CARTESIAN_POINT ( 'NONE',  ( -12.09999999999999609, 12.50000000000000000, 1.734723475976807094E-15 ) ) ;
#28609=DIRECTION ( 'NONE',  ( -0.000000000000000000, 1.000000000000000000, -0.000000000000000000 ) ) ;
#28610=DIRECTION ( 'NONE',  ( 0.000000000000000000, 1.000000000000000000, 0.000000000000000000 ) ) ;
#28611=DIRECTION ( 'NONE',  ( -0.000000000000000000, 1.000000000000000000, -0.000000000000000000 ) ) ;
#28612=EDGE_CURVE ( 'NONE', #67778, #28988, #10921, .T. ) ;
#28613=EDGE_LOOP ( 'NONE', ( #103172, #86716 ) ) ;
#28614=CARTESIAN_POINT ( 'NONE',  ( -9.800000000000004263, 2.500000000000000000, 4.083716857408420609 ) ) ;
#28615=DIRECTION ( 'NONE',  ( -0.000000000000000000, 1.000000000000000000, -0.000000000000000000 ) ) ;
#28616=DIRECTION ( 'NONE',  ( 0.000000000000000000, -0.9999939076577903929, 0.003490651415223739937 ) ) ;
#28617=ORIENTED_EDGE ( 'NONE', *, *, #78517, .F. ) ;
#28618=AXIS2_PLACEMENT_3D ( 'NONE', #99863, #38374, #118203 ) ;
#28619=AXIS2_PLACEMENT_3D ( 'NONE', #17725, #34834, #24986 ) ;
#28620=EDGE_LOOP ( 'NONE', ( #5390, #93627 ) ) ;
#28621=AXIS2_PLACEMENT_3D ( 'NONE', #66347, #95817, #45439 ) ;
#28622=CARTESIAN_POINT ( 'NONE',  ( 0.4499999999999573785, 12.50000000000000000, -6.560283801567339701 ) ) ;
#28623=CIRCLE ( 'NONE', #68320, 0.06509327318403745899 ) ;
#28624=ORIENTED_EDGE ( 'NONE', *, *, #103970, .F. ) ;
#28625=ORIENTED_EDGE ( 'NONE', *, *, #122340, .F. ) ;
#28626=EDGE_LOOP ( 'NONE', ( #17498, #63702, #87939, #75727 ) ) ;
#28627=CARTESIAN_POINT ( 'NONE',  ( 8.349999999999923261, 2.500000000000000000, 2.065063509461097624 ) ) ;
#28628=AXIS2_PLACEMENT_3D ( 'NONE', #129479, #30623, #20144 ) ;
#28629=CARTESIAN_POINT ( 'NONE',  ( 3.099999999999944134, 12.50000000000000000, 4.741630453620009789 ) ) ;
#28630=CARTESIAN_POINT ( 'NONE',  ( -8.749999999999975131, 12.50000000000000000, -2.230156782645139391 ) ) ;
#28631=AXIS2_PLACEMENT_3D ( 'NONE', #79700, #41096, #110446 ) ;
#28632=DIRECTION ( 'NONE',  ( 0.000000000000000000, 0.000000000000000000, -1.000000000000000000 ) ) ;
#28633=ORIENTED_EDGE ( 'NONE', *, *, #7323, .F. ) ;
#28634=CONICAL_SURFACE ( 'NONE', #124768, 0.09999999999999982514, 0.003490658503988666988 ) ;
#28635=DIRECTION ( 'NONE',  ( 0.000000000000000000, -0.000000000000000000, 1.000000000000000000 ) ) ;
#28636=ORIENTED_EDGE ( 'NONE', *, *, #65318, .F. ) ;
#28637=FACE_OUTER_BOUND ( 'NONE', #107858, .T. ) ;
#28638=CARTESIAN_POINT ( 'NONE',  ( 16.68526679983500571, -0.4774970013481819042, -5.954360761643378019 ) ) ;
#28639=CARTESIAN_POINT ( 'NONE',  ( 20.69433222467986511, 2.585316282074592298, 4.139109617386874440 ) ) ;
#28640=CARTESIAN_POINT ( 'NONE',  ( -2.500000000000031086, 12.50000000000000000, 3.702399969078682407 ) ) ;
#28641=AXIS2_PLACEMENT_3D ( 'NONE', #122409, #71346, #30818 ) ;
#28642=DIRECTION ( 'NONE',  ( 0.000000000000000000, 0.000000000000000000, -1.000000000000000000 ) ) ;
#28643=AXIS2_PLACEMENT_3D ( 'NONE', #55056, #84514, #34788 ) ;
#28644=VERTEX_POINT ( 'NONE', #117074 ) ;
#28645=EDGE_CURVE ( 'NONE', #76002, #18774, #42356, .T. ) ;
#28646=AXIS2_PLACEMENT_3D ( 'NONE', #128045, #18079, #18731 ) ;
#28647=AXIS2_PLACEMENT_3D ( 'NONE', #64103, #124318, #86307 ) ;
#28648=ORIENTED_EDGE ( 'NONE', *, *, #128049, .T. ) ;
#28649=ORIENTED_EDGE ( 'NONE', *, *, #59533, .T. ) ;
#28650=VERTEX_POINT ( 'NONE', #124984 ) ;
#28651=ADVANCED_FACE ( 'NONE', ( #35326 ), #69523, .T. ) ;
#28652=ORIENTED_EDGE ( 'NONE', *, *, #119586, .T. ) ;
#28653=DIRECTION ( 'NONE',  ( -0.000000000000000000, 1.000000000000000000, -0.000000000000000000 ) ) ;
#28654=CARTESIAN_POINT ( 'NONE',  ( -8.950000000000006395, 2.500000000000000000, 6.941600689897073018 ) ) ;
#28655=CARTESIAN_POINT ( 'NONE',  ( -7.900000000000014566, 2.500000000000000000, -0.6928203230275541413 ) ) ;
#28656=FACE_BOUND ( 'NONE', #31140, .T. ) ;
#28657=CARTESIAN_POINT ( 'NONE',  ( -12.49999999999999289, 12.50000000000000000, -5.022947341949751454 ) ) ;
#28658=DIRECTION ( 'NONE',  ( 0.000000000000000000, 0.000000000000000000, 1.000000000000000000 ) ) ;
#28659=CARTESIAN_POINT ( 'NONE',  ( 10.64999999999990976, 2.500000000000000000, 2.511473670974873507 ) ) ;
#28660=FACE_OUTER_BOUND ( 'NONE', #92443, .T. ) ;
#28662=FACE_OUTER_BOUND ( 'NONE', #117299, .T. ) ;
#28663=AXIS2_PLACEMENT_3D ( 'NONE', #66516, #106451, #9551 ) ;
#28664=CARTESIAN_POINT ( 'NONE',  ( -5.850000000000021849, 2.500000000000000000, -5.902370205355750521 ) ) ;
#28665=FACE_OUTER_BOUND ( 'NONE', #66934, .T. ) ;
#28666=ORIENTED_EDGE ( 'NONE', *, *, #97314, .F. ) ;
#28667=ORIENTED_EDGE ( 'NONE', *, *, #53376, .T. ) ;
#28668=ORIENTED_EDGE ( 'NONE', *, *, #79452, .F. ) ;
#28669=EDGE_LOOP ( 'NONE', ( #33444, #33858, #76679, #120271 ) ) ;
#28670=DIRECTION ( 'NONE',  ( 0.000000000000000000, 0.000000000000000000, -1.000000000000000000 ) ) ;
#28671=CARTESIAN_POINT ( 'NONE',  ( -8.550000000000013145, 2.500000000000000000, 2.511473670974873507 ) ) ;
#28672=FACE_BOUND ( 'NONE', #6641, .T. ) ;
#28673=CARTESIAN_POINT ( 'NONE',  ( 12.49999999999993960, 2.500000000000000000, 4.230127018922196669 ) ) ;
#28674=CONICAL_SURFACE ( 'NONE', #97620, 0.1000000000000002554, 0.003490658503988666988 ) ;
#28675=AXIS2_PLACEMENT_3D ( 'NONE', #83038, #94126, #122951 ) ;
#28676=VERTEX_POINT ( 'NONE', #109195 ) ;
#28677=DIRECTION ( 'NONE',  ( 0.000000000000000000, -0.000000000000000000, 1.000000000000000000 ) ) ;
#28678=CARTESIAN_POINT ( 'NONE',  ( 9.399999999999915090, 2.500000000000000000, 4.776537180435972196 ) ) ;
#28679=DIRECTION ( 'NONE',  ( 0.000000000000000000, 0.000000000000000000, 1.000000000000000000 ) ) ;
#28680=LINE ( 'NONE', #70523, #43221 ) ;
#28682=DIRECTION ( 'NONE',  ( 0.000000000000000000, 0.000000000000000000, -1.000000000000000000 ) ) ;
#28683=VECTOR ( 'NONE', #71274, 1000.000000000000000 ) ;
#28684=VECTOR ( 'NONE', #1870, 1000.000000000000000 ) ;
#28685=ADVANCED_FACE ( 'NONE', ( #109864 ), #79912, .T. ) ;
#28686=ORIENTED_EDGE ( 'NONE', *, *, #26729, .T. ) ;
#28687=ORIENTED_EDGE ( 'NONE', *, *, #29076, .T. ) ;
#28688=DIRECTION ( 'NONE',  ( -0.000000000000000000, 1.000000000000000000, -0.000000000000000000 ) ) ;
#28689=DIRECTION ( 'NONE',  ( 0.000000000000000000, 1.000000000000000000, 0.000000000000000000 ) ) ;
#28691=CIRCLE ( 'NONE', #126887, 0.1000000000000002554 ) ;
#28692=CONICAL_SURFACE ( 'NONE', #83077, 0.1000000000000002554, 0.003490658503988666988 ) ;
#28693=VECTOR ( 'NONE', #65534, 1000.000000000000000 ) ;
#28694=DIRECTION ( 'NONE',  ( 0.000000000000000000, 0.000000000000000000, -1.000000000000000000 ) ) ;
#28695=DIRECTION ( 'NONE',  ( -0.000000000000000000, 1.000000000000000000, -0.000000000000000000 ) ) ;
#28696=EDGE_LOOP ( 'NONE', ( #127600, #36920 ) ) ;
#28697=CARTESIAN_POINT ( 'NONE',  ( 9.349999999999916156, 12.50000000000000000, 6.841600689897072485 ) ) ;
#28698=ORIENTED_EDGE ( 'NONE', *, *, #77817, .F. ) ;
#28699=EDGE_CURVE ( 'NONE', #29893, #81561, #86240, .T. ) ;
#28700=ADVANCED_FACE ( 'NONE', ( #110495 ), #86143, .T. ) ;
#28701=DIRECTION ( 'NONE',  ( -0.000000000000000000, -1.000000000000000000, -0.000000000000000000 ) ) ;
#28702=ORIENTED_EDGE ( 'NONE', *, *, #124157, .F. ) ;
#28704=FACE_BOUND ( 'NONE', #95949, .T. ) ;
#28705=ORIENTED_EDGE ( 'NONE', *, *, #29806, .F. ) ;
#28708=DIRECTION ( 'NONE',  ( 0.000000000000000000, 0.000000000000000000, -1.000000000000000000 ) ) ;
#28710=DIRECTION ( 'NONE',  ( 0.000000000000000000, 0.000000000000000000, 1.000000000000000000 ) ) ;
#28711=CARTESIAN_POINT ( 'NONE',  ( 6.449999999999930012, 2.500000000000000000, -1.818653347947326138 ) ) ;
#28712=ADVANCED_FACE ( 'NONE', ( #69934 ), #31889, .T. ) ;
#28713=FACE_OUTER_BOUND ( 'NONE', #21622, .T. ) ;
#28714=CIRCLE ( 'NONE', #16064, 0.1000000000000000472 ) ;
#28715=ORIENTED_EDGE ( 'NONE', *, *, #120658, .T. ) ;
#28716=AXIS2_PLACEMENT_3D ( 'NONE', #51883, #32259, #12577 ) ;
#28717=ORIENTED_EDGE ( 'NONE', *, *, #96807, .T. ) ;
#28718=ORIENTED_EDGE ( 'NONE', *, *, #64341, .F. ) ;
#28719=DIRECTION ( 'NONE',  ( 0.000000000000000000, 0.000000000000000000, -1.000000000000000000 ) ) ;
#28720=AXIS2_PLACEMENT_3D ( 'NONE', #42817, #61140, #2199 ) ;
#28721=DIRECTION ( 'NONE',  ( -0.000000000000000000, 1.000000000000000000, -0.000000000000000000 ) ) ;
#28722=DIRECTION ( 'NONE',  ( 0.000000000000000000, 0.000000000000000000, 1.000000000000000000 ) ) ;
#28723=VERTEX_POINT ( 'NONE', #10363 ) ;
#28724=EDGE_LOOP ( 'NONE', ( #58205, #61746 ) ) ;
#28725=ORIENTED_EDGE ( 'NONE', *, *, #112419, .T. ) ;
#28726=DIRECTION ( 'NONE',  ( -0.000000000000000000, 1.000000000000000000, -0.000000000000000000 ) ) ;
#28727=VECTOR ( 'NONE', #63128, 1000.000000000000000 ) ;
#28728=CONICAL_SURFACE ( 'NONE', #93472, 0.1000000000000002554, 0.003490658503988666988 ) ;
#28729=DIRECTION ( 'NONE',  ( 0.000000000000000000, -0.000000000000000000, 1.000000000000000000 ) ) ;
#28731=PLANE ( 'NONE',  #90816 ) ;
#28732=DIRECTION ( 'NONE',  ( 0.000000000000000000, 1.000000000000000000, 0.000000000000000000 ) ) ;
#28733=DIRECTION ( 'NONE',  ( -4.274815082592931898E-19, -0.9999939076577903929, -0.003490651415223739937 ) ) ;
#28734=CARTESIAN_POINT ( 'NONE',  ( 6.899999999999928413, 2.500000000000000000, 4.083716857408421497 ) ) ;
#28735=DIRECTION ( 'NONE',  ( -0.000000000000000000, -1.000000000000000000, -0.000000000000000000 ) ) ;
#28736=CARTESIAN_POINT ( 'NONE',  ( 3.349999999999941913, 2.500000000000000000, 6.495190528383297135 ) ) ;
#28737=ORIENTED_EDGE ( 'NONE', *, *, #50474, .F. ) ;
#28738=VERTEX_POINT ( 'NONE', #90192 ) ;
#28739=EDGE_CURVE ( 'NONE', #13047, #49424, #28077, .T. ) ;
#28740=CARTESIAN_POINT ( 'NONE',  ( 1.849999999999951017, 12.50000000000000000, -6.148780366869526226 ) ) ;
#28741=CIRCLE ( 'NONE', #39228, 0.06509327318403745899 ) ;
#28742=CONICAL_SURFACE ( 'NONE', #106090, 0.09999999999999982514, 0.003490658503988666988 ) ;
#28743=CARTESIAN_POINT ( 'NONE',  ( -0.6500000000000394351, 2.500000000000000000, 6.741600689897071952 ) ) ;
#28744=EDGE_LOOP ( 'NONE', ( #70108, #126424, #52314, #28511 ) ) ;
#28745=EDGE_LOOP ( 'NONE', ( #106457, #77903, #11849, #108449 ) ) ;
#28746=ADVANCED_FACE ( 'NONE', ( #49022 ), #20189, .T. ) ;
#28748=DIRECTION ( 'NONE',  ( 0.000000000000000000, 1.000000000000000000, 0.000000000000000000 ) ) ;
#28749=DIRECTION ( 'NONE',  ( 0.000000000000000000, 1.000000000000000000, 0.000000000000000000 ) ) ;
#28750=ADVANCED_FACE ( 'NONE', ( #88256 ), #54851, .T. ) ;
#28751=DIRECTION ( 'NONE',  ( 0.000000000000000000, 0.000000000000000000, -1.000000000000000000 ) ) ;
#28752=CARTESIAN_POINT ( 'NONE',  ( -12.89999999999999147, 2.500000000000000000, -4.330127018922198978 ) ) ;
#28753=LINE ( 'NONE', #37913, #19744 ) ;
#28754=CARTESIAN_POINT ( 'NONE',  ( -9.400000000000007461, 2.500000000000000000, 4.676537180435972552 ) ) ;
#28755=EDGE_CURVE ( 'NONE', #13760, #88783, #44403, .T. ) ;
#28757=EDGE_CURVE ( 'NONE', #16470, #23090, #40205, .T. ) ;
#28758=CIRCLE ( 'NONE', #118620, 0.09999999999999982514 ) ;
#28759=EDGE_CURVE ( 'NONE', #127685, #71566, #37889, .T. ) ;
#28760=DIRECTION ( 'NONE',  ( 0.000000000000000000, 0.000000000000000000, 1.000000000000000000 ) ) ;
#28762=ORIENTED_EDGE ( 'NONE', *, *, #119498, .F. ) ;
#28763=ADVANCED_FACE ( 'NONE', ( #129527 ), #36087, .T. ) ;
#28764=EDGE_LOOP ( 'NONE', ( #39334, #103957 ) ) ;
#28765=ORIENTED_EDGE ( 'NONE', *, *, #35514, .F. ) ;
#28766=EDGE_LOOP ( 'NONE', ( #65585, #114699 ) ) ;
#28767=CARTESIAN_POINT ( 'NONE',  ( 3.099999999999945466, 12.50000000000000000, -4.048810130592463530 ) ) ;
#28768=CARTESIAN_POINT ( 'NONE',  ( 8.349999999999923261, 12.50000000000000000, 1.407149913249508000 ) ) ;
#28769=ADVANCED_FACE ( 'NONE', ( #128219 ), #38564, .T. ) ;
#28770=ORIENTED_EDGE ( 'NONE', *, *, #125485, .T. ) ;
#28771=CIRCLE ( 'NONE', #116572, 0.06509327318403745899 ) ;
#28773=VECTOR ( 'NONE', #94443, 1000.000000000000000 ) ;
#28774=DIRECTION ( 'NONE',  ( -0.000000000000000000, -1.000000000000000000, -0.000000000000000000 ) ) ;
#28775=DIRECTION ( 'NONE',  ( 0.000000000000000000, 1.000000000000000000, 0.000000000000000000 ) ) ;
#28776=DIRECTION ( 'NONE',  ( 0.000000000000000000, 0.000000000000000000, 1.000000000000000000 ) ) ;
#28777=VERTEX_POINT ( 'NONE', #108566 ) ;
#28778=DIRECTION ( 'NONE',  ( 0.000000000000000000, 1.000000000000000000, 0.000000000000000000 ) ) ;
#28779=AXIS2_PLACEMENT_3D ( 'NONE', #80317, #433, #8331 ) ;
#28780=LINE ( 'NONE', #30729, #58279 ) ;
#28781=ORIENTED_EDGE ( 'NONE', *, *, #52122, .F. ) ;
#28782=AXIS2_PLACEMENT_3D ( 'NONE', #15159, #66212, #106148 ) ;
#28783=ORIENTED_EDGE ( 'NONE', *, *, #96532, .F. ) ;
#28784=ORIENTED_EDGE ( 'NONE', *, *, #10418, .T. ) ;
#28785=FACE_OUTER_BOUND ( 'NONE', #64148, .T. ) ;
#28786=CIRCLE ( 'NONE', #80737, 0.06509327318403745899 ) ;
#28787=DIRECTION ( 'NONE',  ( 0.000000000000000000, 0.000000000000000000, -1.000000000000000000 ) ) ;
#28788=CIRCLE ( 'NONE', #116503, 0.1000000000000002554 ) ;
#28789=ORIENTED_EDGE ( 'NONE', *, *, #10381, .T. ) ;
#28790=AXIS2_PLACEMENT_3D ( 'NONE', #61924, #102476, #71729 ) ;
#28791=CARTESIAN_POINT ( 'NONE',  ( 9.149999999999916866, 2.500000000000000000, -1.572243186433550211 ) ) ;
#28792=CARTESIAN_POINT ( 'NONE',  ( -7.950000000000009059, 12.50000000000000000, 6.495190528383297135 ) ) ;
#28793=DIRECTION ( 'NONE',  ( 0.000000000000000000, 1.000000000000000000, 0.000000000000000000 ) ) ;
#28794=CARTESIAN_POINT ( 'NONE',  ( 13.14999999999989733, 2.500000000000000000, -1.718653347947325827 ) ) ;
#28795=EDGE_LOOP ( 'NONE', ( #91325, #61306 ) ) ;
#28796=CIRCLE ( 'NONE', #14101, 0.06509327318403745899 ) ;
#28797=DIRECTION ( 'NONE',  ( 0.000000000000000000, 1.000000000000000000, 0.000000000000000000 ) ) ;
#28798=ADVANCED_FACE ( 'NONE', ( #98730 ), #128029, .T. ) ;
#28799=AXIS2_PLACEMENT_3D ( 'NONE', #58959, #82313, #112412 ) ;
#28800=ORIENTED_EDGE ( 'NONE', *, *, #128811, .T. ) ;
#28801=EDGE_LOOP ( 'NONE', ( #121129, #30949, #56469, #29171 ) ) ;
#28802=CARTESIAN_POINT ( 'NONE',  ( 7.949999999999922018, 2.500000000000000000, 6.495190528383297135 ) ) ;
#28803=DIRECTION ( 'NONE',  ( 0.000000000000000000, 1.000000000000000000, 0.000000000000000000 ) ) ;
#28804=FACE_BOUND ( 'NONE', #91141, .T. ) ;
#28805=CIRCLE ( 'NONE', #20394, 0.1000000000000002554 ) ;
#28806=DIRECTION ( 'NONE',  ( 0.000000000000000000, 0.000000000000000000, -1.000000000000000000 ) ) ;
#28807=CARTESIAN_POINT ( 'NONE',  ( -2.900000000000029221, 12.50000000000000000, -4.330127018922201643 ) ) ;
#28808=CIRCLE ( 'NONE', #68501, 0.09999999999999999167 ) ;
#28809=CARTESIAN_POINT ( 'NONE',  ( 2.049999999999950084, 12.50000000000000000, -6.560283801567339701 ) ) ;
#28811=AXIS2_PLACEMENT_3D ( 'NONE', #112822, #51341, #924 ) ;
#28812=ORIENTED_EDGE ( 'NONE', *, *, #78583, .T. ) ;
#28813=DIRECTION ( 'NONE',  ( 0.000000000000000000, 1.000000000000000000, 0.000000000000000000 ) ) ;
#28814=CARTESIAN_POINT ( 'NONE',  ( -4.076600168545496672E-14, 12.50000000000000000, -5.022947341949754119 ) ) ;
#28815=CIRCLE ( 'NONE', #101971, 0.06509327318403745899 ) ;
#28816=CARTESIAN_POINT ( 'NONE',  ( 5.849999999999935696, 2.500000000000000000, -6.495190528383302464 ) ) ;
#28817=CIRCLE ( 'NONE', #101972, 0.06509327318403745899 ) ;
#28818=DIRECTION ( 'NONE',  ( 0.000000000000000000, 0.000000000000000000, 1.000000000000000000 ) ) ;
#28819=ORIENTED_EDGE ( 'NONE', *, *, #114950, .T. ) ;
#28820=CARTESIAN_POINT ( 'NONE',  ( -2.700000000000030820, 12.50000000000000000, -3.983716857408426293 ) ) ;
#28821=AXIS2_PLACEMENT_3D ( 'NONE', #69333, #70005, #41844 ) ;
#28822=DIRECTION ( 'NONE',  ( 0.000000000000000000, 0.000000000000000000, 1.000000000000000000 ) ) ;
#28823=EDGE_LOOP ( 'NONE', ( #66001, #21890 ) ) ;
#28824=ORIENTED_EDGE ( 'NONE', *, *, #799, .F. ) ;
#28825=CARTESIAN_POINT ( 'NONE',  ( 9.149999999999915090, 2.500000000000000000, -2.265063509461101798 ) ) ;
#28827=DIRECTION ( 'NONE',  ( -4.274815082592931898E-19, -0.9999939076577903929, -0.003490651415223739937 ) ) ;
#28828=FACE_BOUND ( 'NONE', #85215, .T. ) ;
#28829=CARTESIAN_POINT ( 'NONE',  ( 8.349999999999923261, 12.50000000000000000, 1.472243186433545459 ) ) ;
#28830=CIRCLE ( 'NONE', #39318, 0.1000000000000002554 ) ;
#28831=CIRCLE ( 'NONE', #101989, 0.06509327318403745899 ) ;
#28832=ORIENTED_EDGE ( 'NONE', *, *, #55932, .T. ) ;
#28833=DIRECTION ( 'NONE',  ( 0.000000000000000000, 1.000000000000000000, 0.000000000000000000 ) ) ;
#28834=ORIENTED_EDGE ( 'NONE', *, *, #21191, .F. ) ;
#28835=ORIENTED_EDGE ( 'NONE', *, *, #126582, .F. ) ;
#28836=DIRECTION ( 'NONE',  ( -0.000000000000000000, -1.000000000000000000, -0.000000000000000000 ) ) ;
#28838=ORIENTED_EDGE ( 'NONE', *, *, #57612, .T. ) ;
#28839=DIRECTION ( 'NONE',  ( 0.000000000000000000, 0.000000000000000000, -1.000000000000000000 ) ) ;
#28840=DIRECTION ( 'NONE',  ( -0.000000000000000000, -1.000000000000000000, -0.000000000000000000 ) ) ;
#28841=EDGE_CURVE ( 'NONE', #36170, #100170, #565, .T. ) ;
#28842=FACE_OUTER_BOUND ( 'NONE', #44177, .T. ) ;
#28844=ADVANCED_FACE ( 'NONE', ( #1187 ), #100911, .T. ) ;
#28845=ORIENTED_EDGE ( 'NONE', *, *, #111728, .F. ) ;
#28847=CARTESIAN_POINT ( 'NONE',  ( 6.449999999999930012, 2.500000000000000000, 1.918653347947321564 ) ) ;
#28849=CARTESIAN_POINT ( 'NONE',  ( 2.299999999999948752, 2.500000000000000000, -4.083716857408426826 ) ) ;
#28850=ORIENTED_EDGE ( 'NONE', *, *, #44877, .T. ) ;
#28852=EDGE_CURVE ( 'NONE', #92706, #64742, #98861, .T. ) ;
#28853=ORIENTED_EDGE ( 'NONE', *, *, #125628, .F. ) ;
#28854=EDGE_CURVE ( 'NONE', #84759, #93988, #8973, .T. ) ;
#28855=CARTESIAN_POINT ( 'NONE',  ( -8.750000000000005329, 2.500000000000000000, 5.802370205355744659 ) ) ;
#28856=EDGE_LOOP ( 'NONE', ( #98669, #71943 ) ) ;
#28857=DIRECTION ( 'NONE',  ( 0.000000000000000000, 0.000000000000000000, 1.000000000000000000 ) ) ;
#28858=CARTESIAN_POINT ( 'NONE',  ( 5.849999999999935696, 2.500000000000000000, -6.495190528383302464 ) ) ;
#28859=AXIS2_PLACEMENT_3D ( 'NONE', #114672, #96315, #86500 ) ;
#28860=DIRECTION ( 'NONE',  ( 0.000000000000000000, 0.000000000000000000, -1.000000000000000000 ) ) ;
#28861=AXIS2_PLACEMENT_3D ( 'NONE', #119247, #38788, #19770 ) ;
#28862=DIRECTION ( 'NONE',  ( 0.000000000000000000, 1.000000000000000000, 0.000000000000000000 ) ) ;
#28863=ORIENTED_EDGE ( 'NONE', *, *, #105256, .T. ) ;
#28864=ADVANCED_FACE ( 'NONE', ( #113065 ), #122905, .T. ) ;
#28865=DIRECTION ( 'NONE',  ( 0.000000000000000000, -0.9999939076577903929, 0.003490651415223739937 ) ) ;
#28866=DIRECTION ( 'NONE',  ( -0.000000000000000000, -1.000000000000000000, -0.000000000000000000 ) ) ;
#28867=CARTESIAN_POINT ( 'NONE',  ( 81.97672699151137010, 3.779183617727026601, -6.223416210580854369 ) ) ;
#28869=DIRECTION ( 'NONE',  ( 0.000000000000000000, -0.9999939076577903929, 0.003490651415223739937 ) ) ;
#28870=EDGE_CURVE ( 'NONE', #60531, #59400, #52232, .T. ) ;
#28871=LINE ( 'NONE', #7267, #122655 ) ;
#28872=VECTOR ( 'NONE', #48055, 1000.000000000000000 ) ;
#28873=VERTEX_POINT ( 'NONE', #52872 ) ;
#28874=CIRCLE ( 'NONE', #47744, 0.09999999999999999167 ) ;
#28875=ORIENTED_EDGE ( 'NONE', *, *, #50072, .F. ) ;
#28876=PLANE ( 'NONE',  #108039 ) ;
#28877=VERTEX_POINT ( 'NONE', #1822 ) ;
#28879=ORIENTED_EDGE ( 'NONE', *, *, #115159, .T. ) ;
#28880=ORIENTED_EDGE ( 'NONE', *, *, #97849, .T. ) ;
#28881=EDGE_LOOP ( 'NONE', ( #119986, #129128, #126555, #119816 ) ) ;
#28882=DIRECTION ( 'NONE',  ( -0.000000000000000000, -1.000000000000000000, -0.000000000000000000 ) ) ;
#28883=VECTOR ( 'NONE', #56353, 1000.000000000000000 ) ;
#28884=FACE_OUTER_BOUND ( 'NONE', #18578, .T. ) ;
#28885=CARTESIAN_POINT ( 'NONE',  ( -3.550000000000030909, 12.50000000000000000, -6.906693963081115939 ) ) ;
#28886=DIRECTION ( 'NONE',  ( 0.000000000000000000, 1.000000000000000000, 0.000000000000000000 ) ) ;
#28887=DIRECTION ( 'NONE',  ( 0.000000000000000000, 0.000000000000000000, 1.000000000000000000 ) ) ;
#28888=CARTESIAN_POINT ( 'NONE',  ( -7.700000000000010836, 12.50000000000000000, 3.918623584224383727 ) ) ;
#28889=CIRCLE ( 'NONE', #10000, 2.000000000000000000 ) ;
#28890=CARTESIAN_POINT ( 'NONE',  ( 2.299999999999946976, 2.500000000000000000, 4.576537180435972019 ) ) ;
#28891=CARTESIAN_POINT ( 'NONE',  ( -6.050000000000022027, 12.50000000000000000, -1.818653347947326138 ) ) ;
#28892=ORIENTED_EDGE ( 'NONE', *, *, #71468, .F. ) ;
#28893=VECTOR ( 'NONE', #100902, 1000.000000000000000 ) ;
#28894=ORIENTED_EDGE ( 'NONE', *, *, #89940, .F. ) ;
#28895=EDGE_LOOP ( 'NONE', ( #56588, #61210 ) ) ;
#28896=AXIS2_PLACEMENT_3D ( 'NONE', #80064, #118044, #9395 ) ;
#28898=VERTEX_POINT ( 'NONE', #112445 ) ;
#28899=ORIENTED_EDGE ( 'NONE', *, *, #23201, .T. ) ;
#28900=CARTESIAN_POINT ( 'NONE',  ( -13.74999999999998757, 2.500000000000000000, -2.757883832488651876 ) ) ;
#28901=CIRCLE ( 'NONE', #106165, 0.06509327318403745899 ) ;
#28902=AXIS2_PLACEMENT_3D ( 'NONE', #43865, #53030, #102126 ) ;
#28903=EDGE_CURVE ( 'NONE', #62546, #115890, #119699, .T. ) ;
#28904=DIRECTION ( 'NONE',  ( 0.000000000000000000, 0.000000000000000000, -1.000000000000000000 ) ) ;
#28905=CONICAL_SURFACE ( 'NONE', #18513, 0.1000000000000002554, 0.003490658503988666988 ) ;
#28906=DIRECTION ( 'NONE',  ( 0.000000000000000000, 1.000000000000000000, 0.000000000000000000 ) ) ;
#28907=CARTESIAN_POINT ( 'NONE',  ( -11.64999999999999858, 2.500000000000000000, -5.802370205355746435 ) ) ;
#28908=EDGE_CURVE ( 'NONE', #125626, #117945, #40305, .T. ) ;
#28909=CARTESIAN_POINT ( 'NONE',  ( -1.650000000000034772, 12.50000000000000000, 2.165063509461097713 ) ) ;
#28910=VERTEX_POINT ( 'NONE', #100661 ) ;
#28911=ADVANCED_FACE ( 'NONE', ( #31951 ), #63272, .T. ) ;
#28912=AXIS2_PLACEMENT_3D ( 'NONE', #13867, #32255, #53798 ) ;
#28913=ADVANCED_FACE ( 'NONE', ( #41137 ), #92616, .T. ) ;
#28914=EDGE_CURVE ( 'NONE', #109859, #94650, #121849, .T. ) ;
#28915=ORIENTED_EDGE ( 'NONE', *, *, #21180, .T. ) ;
#28916=LINE ( 'NONE', #27590, #30010 ) ;
#28917=EDGE_LOOP ( 'NONE', ( #25837, #124605 ) ) ;
#28918=CARTESIAN_POINT ( 'NONE',  ( 6.049999999999934097, 2.500000000000000000, -2.511473670974877948 ) ) ;
#28919=ADVANCED_FACE ( 'NONE', ( #2456 ), #54956, .T. ) ;
#28920=ORIENTED_EDGE ( 'NONE', *, *, #94496, .F. ) ;
#28921=CONICAL_SURFACE ( 'NONE', #104123, 0.1000000000000002554, 0.003490658503988666988 ) ;
#28922=ORIENTED_EDGE ( 'NONE', *, *, #91843, .F. ) ;
#28923=DIRECTION ( 'NONE',  ( -0.000000000000000000, -1.000000000000000000, -0.000000000000000000 ) ) ;
#28924=DIRECTION ( 'NONE',  ( 0.000000000000000000, 0.000000000000000000, 1.000000000000000000 ) ) ;
#28925=EDGE_CURVE ( 'NONE', #112846, #32323, #4758, .T. ) ;
#28926=AXIS2_PLACEMENT_3D ( 'NONE', #81065, #87794, #31327 ) ;
#28927=ADVANCED_FACE ( 'NONE', ( #42417 ), #51595, .T. ) ;
#28928=LINE ( 'NONE', #68832, #59187 ) ;
#28929=DIRECTION ( 'NONE',  ( 0.000000000000000000, 0.000000000000000000, 1.000000000000000000 ) ) ;
#28930=CARTESIAN_POINT ( 'NONE',  ( -5.400000000000023448, 2.500000000000000000, -5.022947341949754119 ) ) ;
#28931=VERTEX_POINT ( 'NONE', #61418 ) ;
#28932=DIRECTION ( 'NONE',  ( 0.000000000000000000, -0.9999939076577903929, 0.003490651415223739937 ) ) ;
#28933=CARTESIAN_POINT ( 'NONE',  ( -10.65000000000000213, 12.50000000000000000, 2.446380397790835826 ) ) ;
#28934=PLANE ( 'NONE',  #83381 ) ;
#28935=DIRECTION ( 'NONE',  ( -0.000000000000000000, 1.000000000000000000, -0.000000000000000000 ) ) ;
#28936=CARTESIAN_POINT ( 'NONE',  ( -1.650000000000034328, 12.50000000000000000, -6.495190528383302464 ) ) ;
#28937=ORIENTED_EDGE ( 'NONE', *, *, #31268, .F. ) ;
#28938=ORIENTED_EDGE ( 'NONE', *, *, #52507, .T. ) ;
#28939=CONICAL_SURFACE ( 'NONE', #127233, 0.09999999999999999167, 0.003490658503988666988 ) ;
#28940=CARTESIAN_POINT ( 'NONE',  ( -2.900000000000029221, 2.500000000000000000, -0.1000000000000022815 ) ) ;
#28941=EDGE_CURVE ( 'NONE', #58229, #126385, #72522, .T. ) ;
#28942=VERTEX_POINT ( 'NONE', #129298 ) ;
#28943=FACE_OUTER_BOUND ( 'NONE', #32176, .T. ) ;
#28944=CARTESIAN_POINT ( 'NONE',  ( 6.899999999999928413, 2.500000000000000000, -4.676537180435977881 ) ) ;
#28945=AXIS2_PLACEMENT_3D ( 'NONE', #110067, #79331, #38772 ) ;
#28946=AXIS2_PLACEMENT_3D ( 'NONE', #54639, #84764, #124692 ) ;
#28947=AXIS2_PLACEMENT_3D ( 'NONE', #65388, #75217, #85028 ) ;
#28948=AXIS2_PLACEMENT_3D ( 'NONE', #72029, #121111, #72669 ) ;
#28953=CARTESIAN_POINT ( 'NONE',  ( -9.350000000000006750, 2.500000000000000000, 2.511473670974873507 ) ) ;
#28954=ORIENTED_EDGE ( 'NONE', *, *, #93326, .F. ) ;
#28955=AXIS2_PLACEMENT_3D ( 'NONE', #7274, #107423, #38039 ) ;
#28956=AXIS2_PLACEMENT_3D ( 'NONE', #113226, #85062, #92967 ) ;
#28957=CIRCLE ( 'NONE', #35222, 0.06509327318403745899 ) ;
#28958=CARTESIAN_POINT ( 'NONE',  ( 0.8499999999999553468, 2.500000000000000000, -2.065063509461102065 ) ) ;
#28959=ORIENTED_EDGE ( 'NONE', *, *, #83125, .T. ) ;
#28960=FACE_OUTER_BOUND ( 'NONE', #5665, .T. ) ;
#28961=CARTESIAN_POINT ( 'NONE',  ( -0.4000000000000392131, 12.50000000000000000, -5.022947341949754119 ) ) ;
#28962=CONICAL_SURFACE ( 'NONE', #102113, 0.1000000000000002554, 0.003490658503988666988 ) ;
#28963=CARTESIAN_POINT ( 'NONE',  ( -8.100000000000013856, 2.500000000000000000, -4.676537180435977881 ) ) ;
#28964=EDGE_CURVE ( 'NONE', #117945, #125626, #84192, .T. ) ;
#28965=AXIS2_PLACEMENT_3D ( 'NONE', #106663, #6496, #55638 ) ;
#28966=ORIENTED_EDGE ( 'NONE', *, *, #103566, .F. ) ;
#28967=CARTESIAN_POINT ( 'NONE',  ( 0.8499999999999553468, 2.500000000000000000, 2.165063509461097713 ) ) ;
#28968=ORIENTED_EDGE ( 'NONE', *, *, #62044, .T. ) ;
#28969=DIRECTION ( 'NONE',  ( 0.000000000000000000, -0.000000000000000000, 1.000000000000000000 ) ) ;
#28971=DIRECTION ( 'NONE',  ( 0.000000000000000000, -0.9999939076577903929, 0.003490651415223739937 ) ) ;
#28972=ORIENTED_EDGE ( 'NONE', *, *, #96587, .T. ) ;
#28973=AXIS2_PLACEMENT_3D ( 'NONE', #58162, #47690, #28045 ) ;
#28974=DIRECTION ( 'NONE',  ( 0.000000000000000000, 0.000000000000000000, -1.000000000000000000 ) ) ;
#28975=CARTESIAN_POINT ( 'NONE',  ( 3.749999999999940492, 12.50000000000000000, 5.867463478539781896 ) ) ;
#28976=AXIS2_PLACEMENT_3D ( 'NONE', #47364, #108204, #117348 ) ;
#28977=AXIS2_PLACEMENT_3D ( 'NONE', #36171, #85259, #4105 ) ;
#28978=ORIENTED_EDGE ( 'NONE', *, *, #35816, .F. ) ;
#28979=DIRECTION ( 'NONE',  ( 0.000000000000000000, 0.000000000000000000, -1.000000000000000000 ) ) ;
#28980=EDGE_LOOP ( 'NONE', ( #110484, #126893, #94062, #62642 ) ) ;
#28981=DIRECTION ( 'NONE',  ( 0.000000000000000000, 1.000000000000000000, 0.000000000000000000 ) ) ;
#28982=AXIS2_PLACEMENT_3D ( 'NONE', #18907, #26813, #58850 ) ;
#28983=VERTEX_POINT ( 'NONE', #108959 ) ;
#28985=DIRECTION ( 'NONE',  ( 0.000000000000000000, 0.000000000000000000, 1.000000000000000000 ) ) ;
#28986=LINE ( 'NONE', #96405, #14539 ) ;
#28987=ORIENTED_EDGE ( 'NONE', *, *, #75621, .F. ) ;
#28988=VERTEX_POINT ( 'NONE', #120102 ) ;
#28989=DIRECTION ( 'NONE',  ( 0.000000000000000000, 1.000000000000000000, 0.000000000000000000 ) ) ;
#28990=CARTESIAN_POINT ( 'NONE',  ( -5.600000000000020073, 12.50000000000000000, -0.4115034346978156399 ) ) ;
#28991=CIRCLE ( 'NONE', #41527, 0.06509327318403745899 ) ;
#28992=ORIENTED_EDGE ( 'NONE', *, *, #100030, .F. ) ;
#28993=DIRECTION ( 'NONE',  ( 0.000000000000000000, 0.000000000000000000, 1.000000000000000000 ) ) ;
#28995=CARTESIAN_POINT ( 'NONE',  ( -9.999999999999969802, 12.50000000000000000, 4.265033745738159077 ) ) ;
#28997=FACE_OUTER_BOUND ( 'NONE', #62493, .T. ) ;
#28998=CARTESIAN_POINT ( 'NONE',  ( -14.39999999999998614, 12.50000000000000000, 0.4115034346978132529 ) ) ;
#28999=CARTESIAN_POINT ( 'NONE',  ( -11.44999999999999751, 12.50000000000000000, 1.753560074763284016 ) ) ;
#29000=AXIS2_PLACEMENT_3D ( 'NONE', #111408, #125734, #45920 ) ;
#29001=EDGE_CURVE ( 'NONE', #22580, #13178, #48716, .T. ) ;
#29002=ORIENTED_EDGE ( 'NONE', *, *, #117787, .T. ) ;
#29003=ORIENTED_EDGE ( 'NONE', *, *, #53114, .F. ) ;
#29004=CIRCLE ( 'NONE', #125423, 0.1000000000000002554 ) ;
#29005=EDGE_LOOP ( 'NONE', ( #123437, #74310 ) ) ;
#29006=EDGE_LOOP ( 'NONE', ( #8341, #12888, #31210, #78148 ) ) ;
#29007=DIRECTION ( 'NONE',  ( -0.000000000000000000, -1.000000000000000000, -0.000000000000000000 ) ) ;
#29008=DIRECTION ( 'NONE',  ( 0.000000000000000000, 0.000000000000000000, -1.000000000000000000 ) ) ;
#29009=DIRECTION ( 'NONE',  ( 0.000000000000000000, 1.000000000000000000, 0.000000000000000000 ) ) ;
#29010=CIRCLE ( 'NONE', #12257, 0.06509327318403745899 ) ;
#29011=VERTEX_POINT ( 'NONE', #38993 ) ;
#29012=EDGE_CURVE ( 'NONE', #72399, #3753, #111369, .T. ) ;
#29013=FACE_BOUND ( 'NONE', #13453, .T. ) ;
#29014=VERTEX_POINT ( 'NONE', #69051 ) ;
#29015=ADVANCED_FACE ( 'NONE', ( #69701 ), #107176, .T. ) ;
#29016=LINE ( 'NONE', #68917, #52186 ) ;
#29017=DIRECTION ( 'NONE',  ( 0.000000000000000000, 0.000000000000000000, 1.000000000000000000 ) ) ;
#29018=DIRECTION ( 'NONE',  ( 0.000000000000000000, 1.000000000000000000, 0.000000000000000000 ) ) ;
#29019=AXIS2_PLACEMENT_3D ( 'NONE', #126126, #45652, #106492 ) ;
#29020=LINE ( 'NONE', #77457, #84711 ) ;
#29021=DIRECTION ( 'NONE',  ( 0.000000000000000000, -0.9999939076577903929, 0.003490651415223739937 ) ) ;
#29022=EDGE_CURVE ( 'NONE', #37333, #113704, #99173, .T. ) ;
#29024=EDGE_CURVE ( 'NONE', #32318, #16607, #50762, .T. ) ;
#29025=DIRECTION ( 'NONE',  ( 0.000000000000000000, 1.000000000000000000, 0.000000000000000000 ) ) ;
#29026=CARTESIAN_POINT ( 'NONE',  ( -15.39999999999997904, 2.500000000000000000, 0.1000000000000000056 ) ) ;
#29027=ADVANCED_FACE ( 'NONE', ( #10143 ), #19441, .T. ) ;
#29028=CARTESIAN_POINT ( 'NONE',  ( 14.39999999999989555, 12.50000000000000000, -0.3464101615137782364 ) ) ;
#29029=EDGE_CURVE ( 'NONE', #48878, #98420, #59183, .T. ) ;
#29030=DIRECTION ( 'NONE',  ( 0.000000000000000000, -0.9999939076577903929, 0.003490651415223739937 ) ) ;
#29031=ORIENTED_EDGE ( 'NONE', *, *, #10255, .T. ) ;
#29032=ORIENTED_EDGE ( 'NONE', *, *, #95531, .T. ) ;
#29033=ORIENTED_EDGE ( 'NONE', *, *, #96276, .T. ) ;
#29034=VERTEX_POINT ( 'NONE', #88024 ) ;
#29035=DIRECTION ( 'NONE',  ( 0.000000000000000000, 1.000000000000000000, 0.000000000000000000 ) ) ;
#29036=DIRECTION ( 'NONE',  ( -0.000000000000000000, -1.000000000000000000, -0.000000000000000000 ) ) ;
#29037=ORIENTED_EDGE ( 'NONE', *, *, #42802, .F. ) ;
#29038=ORIENTED_EDGE ( 'NONE', *, *, #27847, .F. ) ;
#29039=EDGE_CURVE ( 'NONE', #90795, #77606, #79995, .T. ) ;
#29040=ORIENTED_EDGE ( 'NONE', *, *, #128407, .T. ) ;
#29041=FACE_OUTER_BOUND ( 'NONE', #88375, .T. ) ;
#29042=AXIS2_PLACEMENT_3D ( 'NONE', #86690, #125332, #97799 ) ;
#29043=LINE ( 'NONE', #108859, #19536 ) ;
#29044=DIRECTION ( 'NONE',  ( 0.000000000000000000, 1.000000000000000000, 0.000000000000000000 ) ) ;
#29045=AXIS2_PLACEMENT_3D ( 'NONE', #110493, #60757, #101970 ) ;
#29046=DIRECTION ( 'NONE',  ( -0.000000000000000000, -1.000000000000000000, -0.000000000000000000 ) ) ;
#29047=CARTESIAN_POINT ( 'NONE',  ( -0.2000000000000347888, 12.50000000000000000, 0.2813168883297384459 ) ) ;
#29048=DIRECTION ( 'NONE',  ( 0.000000000000000000, 1.000000000000000000, 0.000000000000000000 ) ) ;
#29049=DIRECTION ( 'NONE',  ( -0.000000000000000000, -1.000000000000000000, -0.000000000000000000 ) ) ;
#29050=ORIENTED_EDGE ( 'NONE', *, *, #112109, .F. ) ;
#29051=VECTOR ( 'NONE', #126641, 1000.000000000000000 ) ;
#29052=AXIS2_PLACEMENT_3D ( 'NONE', #28736, #98103, #68645 ) ;
#29053=FACE_OUTER_BOUND ( 'NONE', #32051, .T. ) ;
#29054=ORIENTED_EDGE ( 'NONE', *, *, #46315, .T. ) ;
#29055=AXIS2_PLACEMENT_3D ( 'NONE', #127410, #88774, #37744 ) ;
#29056=ORIENTED_EDGE ( 'NONE', *, *, #81991, .T. ) ;
#29057=ORIENTED_EDGE ( 'NONE', *, *, #110575, .T. ) ;
#29058=DIRECTION ( 'NONE',  ( 0.000000000000000000, 0.000000000000000000, 1.000000000000000000 ) ) ;
#29059=EDGE_CURVE ( 'NONE', #81664, #72305, #56993, .T. ) ;
#29060=ORIENTED_EDGE ( 'NONE', *, *, #117775, .F. ) ;
#29061=ORIENTED_EDGE ( 'NONE', *, *, #20878, .T. ) ;
#29062=CIRCLE ( 'NONE', #58300, 0.06509327318403745899 ) ;
#29063=DIRECTION ( 'NONE',  ( -4.274815082592931898E-19, -0.9999939076577903929, -0.003490651415223739937 ) ) ;
#29064=CIRCLE ( 'NONE', #102211, 0.06509327318403745899 ) ;
#29065=DIRECTION ( 'NONE',  ( -0.000000000000000000, 1.000000000000000000, -0.000000000000000000 ) ) ;
#29066=FACE_OUTER_BOUND ( 'NONE', #59679, .T. ) ;
#29067=CARTESIAN_POINT ( 'NONE',  ( 14.39999999999989555, 12.50000000000000000, 0.4115034346978110880 ) ) ;
#29068=LINE ( 'NONE', #82518, #81102 ) ;
#29070=ORIENTED_EDGE ( 'NONE', *, *, #17098, .F. ) ;
#29071=EDGE_CURVE ( 'NONE', #87323, #47163, #78253, .T. ) ;
#29072=DIRECTION ( 'NONE',  ( 0.000000000000000000, 0.000000000000000000, 1.000000000000000000 ) ) ;
#29073=AXIS2_PLACEMENT_3D ( 'NONE', #105653, #35624, #65053 ) ;
#29074=ORIENTED_EDGE ( 'NONE', *, *, #18396, .T. ) ;
#29075=DIRECTION ( 'NONE',  ( 0.000000000000000000, 1.000000000000000000, 0.000000000000000000 ) ) ;
#29076=EDGE_CURVE ( 'NONE', #57844, #98275, #17274, .T. ) ;
#29077=ORIENTED_EDGE ( 'NONE', *, *, #87683, .T. ) ;
#29078=DIRECTION ( 'NONE',  ( 0.000000000000000000, 0.000000000000000000, 1.000000000000000000 ) ) ;
#29079=CARTESIAN_POINT ( 'NONE',  ( -8.100000000000010303, 2.500000000000000000, 4.676537180435972552 ) ) ;
#29080=VERTEX_POINT ( 'NONE', #80826 ) ;
#29082=ADVANCED_FACE ( 'NONE', ( #120734 ), #67441, .T. ) ;
#29083=CARTESIAN_POINT ( 'NONE',  ( -1.850000000000033396, 2.500000000000000000, -2.511473670974877948 ) ) ;
#29084=EDGE_LOOP ( 'NONE', ( #40929, #84879, #92190, #102452 ) ) ;
#29086=EDGE_CURVE ( 'NONE', #73329, #83060, #8832, .T. ) ;
#29087=EDGE_CURVE ( 'NONE', #6145, #100851, #128657, .T. ) ;
#29088=CIRCLE ( 'NONE', #85498, 0.09999999999999982514 ) ;
#29089=DIRECTION ( 'NONE',  ( 0.000000000000000000, 1.000000000000000000, 0.000000000000000000 ) ) ;
#29090=VERTEX_POINT ( 'NONE', #23100 ) ;
#29091=VERTEX_POINT ( 'NONE', #5382 ) ;
#29092=DIRECTION ( 'NONE',  ( 0.000000000000000000, 1.000000000000000000, 0.000000000000000000 ) ) ;
#29093=DIRECTION ( 'NONE',  ( 0.000000000000000000, 0.000000000000000000, -1.000000000000000000 ) ) ;
#29094=CARTESIAN_POINT ( 'NONE',  ( 4.599999999999939249, 12.50000000000000000, -3.637306695894650055 ) ) ;
#29095=DIRECTION ( 'NONE',  ( 0.000000000000000000, 0.000000000000000000, 1.000000000000000000 ) ) ;
#29096=AXIS2_PLACEMENT_3D ( 'NONE', #81389, #11342, #110191 ) ;
#29097=ADVANCED_FACE ( 'NONE', ( #34226 ), #43402, .T. ) ;
#29098=AXIS2_PLACEMENT_3D ( 'NONE', #30747, #33152, #109275 ) ;
#29099=DIRECTION ( 'NONE',  ( 0.000000000000000000, -0.000000000000000000, 1.000000000000000000 ) ) ;
#29100=VERTEX_POINT ( 'NONE', #54482 ) ;
#29101=DIRECTION ( 'NONE',  ( 0.000000000000000000, 1.000000000000000000, 0.000000000000000000 ) ) ;
#29102=CIRCLE ( 'NONE', #41628, 0.06509327318403745899 ) ;
#29103=ORIENTED_EDGE ( 'NONE', *, *, #63810, .F. ) ;
#29104=CARTESIAN_POINT ( 'NONE',  ( 9.149999999999920419, 2.500000000000000000, 1.572243186433545548 ) ) ;
#29105=CARTESIAN_POINT ( 'NONE',  ( -5.600000000000023626, 2.500000000000000000, -4.676537180435977881 ) ) ;
#29106=EDGE_LOOP ( 'NONE', ( #116837, #106072, #27312, #32210 ) ) ;
#29107=CONICAL_SURFACE ( 'NONE', #45821, 0.1000000000000002554, 0.003490658503988666988 ) ;
#29108=AXIS2_PLACEMENT_3D ( 'NONE', #43159, #3845, #103991 ) ;
#29109=AXIS2_PLACEMENT_3D ( 'NONE', #97887, #6907, #8215 ) ;
#29110=FACE_OUTER_BOUND ( 'NONE', #70940, .T. ) ;
#29112=DIRECTION ( 'NONE',  ( 0.000000000000000000, 0.000000000000000000, 1.000000000000000000 ) ) ;
#29113=LINE ( 'NONE', #16027, #31344 ) ;
#29114=FACE_OUTER_BOUND ( 'NONE', #31643, .T. ) ;
#29115=ORIENTED_EDGE ( 'NONE', *, *, #57810, .F. ) ;
#29116=AXIS2_PLACEMENT_3D ( 'NONE', #102620, #53542, #94100 ) ;
#29117=VECTOR ( 'NONE', #128782, 1000.000000000000000 ) ;
#29118=CARTESIAN_POINT ( 'NONE',  ( 7.499999999999927169, 2.500000000000000000, 3.637306695894644726 ) ) ;
#29119=CARTESIAN_POINT ( 'NONE',  ( -9.600000000000008527, 2.500000000000000000, -3.637306695894645614 ) ) ;
#29120=DIRECTION ( 'NONE',  ( 0.000000000000000000, 0.000000000000000000, 1.000000000000000000 ) ) ;
#29121=ORIENTED_EDGE ( 'NONE', *, *, #16582, .T. ) ;
#29122=DIRECTION ( 'NONE',  ( -0.000000000000000000, 1.000000000000000000, -0.000000000000000000 ) ) ;
#29123=EDGE_CURVE ( 'NONE', #37856, #100700, #21514, .T. ) ;
#29125=EDGE_LOOP ( 'NONE', ( #58702, #106124, #35774, #7563 ) ) ;
#29126=LINE ( 'NONE', #16679, #94739 ) ;
#29127=AXIS2_PLACEMENT_3D ( 'NONE', #6122, #76174, #113509 ) ;
#29128=ORIENTED_EDGE ( 'NONE', *, *, #18555, .T. ) ;
#29129=FACE_OUTER_BOUND ( 'NONE', #40113, .T. ) ;
#29130=DIRECTION ( 'NONE',  ( -0.000000000000000000, -1.000000000000000000, -0.000000000000000000 ) ) ;
#29131=ORIENTED_EDGE ( 'NONE', *, *, #53530, .T. ) ;
#29132=CARTESIAN_POINT ( 'NONE',  ( 5.849999999999935696, 12.50000000000000000, -6.560283801567339701 ) ) ;
#29133=AXIS2_PLACEMENT_3D ( 'NONE', #71909, #111828, #111149 ) ;
#29134=DIRECTION ( 'NONE',  ( 0.000000000000000000, 0.000000000000000000, 1.000000000000000000 ) ) ;
#29135=EDGE_LOOP ( 'NONE', ( #50413, #89224 ) ) ;
#29137=EDGE_CURVE ( 'NONE', #84308, #103467, #112777, .T. ) ;
#29138=LINE ( 'NONE', #69033, #55073 ) ;
#29139=AXIS2_PLACEMENT_3D ( 'NONE', #23779, #63701, #104263 ) ;
#29140=EDGE_LOOP ( 'NONE', ( #47732, #10786, #86811, #92440 ) ) ;
#29141=AXIS2_PLACEMENT_3D ( 'NONE', #116930, #88103, #128063 ) ;
#29142=CONICAL_SURFACE ( 'NONE', #125273, 0.1000000000000002554, 0.003490658503988666988 ) ;
#29143=ORIENTED_EDGE ( 'NONE', *, *, #97619, .T. ) ;
#29144=ORIENTED_EDGE ( 'NONE', *, *, #90089, .F. ) ;
#29145=DIRECTION ( 'NONE',  ( 0.000000000000000000, 0.000000000000000000, 1.000000000000000000 ) ) ;
#29146=DIRECTION ( 'NONE',  ( -0.000000000000000000, -1.000000000000000000, -0.000000000000000000 ) ) ;
#29147=LINE ( 'NONE', #79524, #58851 ) ;
#29148=FACE_BOUND ( 'NONE', #111594, .T. ) ;
#29149=VERTEX_POINT ( 'NONE', #65595 ) ;
#29150=CIRCLE ( 'NONE', #10261, 0.06509327318403743123 ) ;
#29151=CARTESIAN_POINT ( 'NONE',  ( 9.199999999999915801, 12.50000000000000000, 4.330127018922196314 ) ) ;
#29152=CARTESIAN_POINT ( 'NONE',  ( 7.949999999999925571, 2.500000000000000000, 2.165063509461097713 ) ) ;
#29153=ORIENTED_EDGE ( 'NONE', *, *, #115256, .T. ) ;
#29154=DIRECTION ( 'NONE',  ( 0.000000000000000000, 0.000000000000000000, 1.000000000000000000 ) ) ;
#29156=AXIS2_PLACEMENT_3D ( 'NONE', #45387, #106231, #33626 ) ;
#29157=DIRECTION ( 'NONE',  ( 0.000000000000000000, 1.000000000000000000, 0.000000000000000000 ) ) ;
#29158=CARTESIAN_POINT ( 'NONE',  ( -1.850000000000033840, 2.500000000000000000, 6.841600689897072485 ) ) ;
#29159=CARTESIAN_POINT ( 'NONE',  ( 6.649999999999930189, 12.50000000000000000, 5.802370205355744659 ) ) ;
#29160=FACE_OUTER_BOUND ( 'NONE', #68524, .T. ) ;
#29161=CARTESIAN_POINT ( 'NONE',  ( -0.2000000000000404232, 12.50000000000000000, 3.918623584224383727 ) ) ;
#29162=EDGE_CURVE ( 'NONE', #28223, #15955, #23656, .T. ) ;
#29163=EDGE_LOOP ( 'NONE', ( #122599, #81252, #60775, #61714 ) ) ;
#29164=VERTEX_POINT ( 'NONE', #102942 ) ;
#29165=ORIENTED_EDGE ( 'NONE', *, *, #34059, .T. ) ;
#29166=EDGE_LOOP ( 'NONE', ( #27306, #30586, #76136, #104708 ) ) ;
#29167=ORIENTED_EDGE ( 'NONE', *, *, #28267, .F. ) ;
#29168=AXIS2_PLACEMENT_3D ( 'NONE', #118259, #59376, #29257 ) ;
#29169=CARTESIAN_POINT ( 'NONE',  ( 1.899999999999949507, 12.50000000000000000, 4.048810130592458201 ) ) ;
#29170=DIRECTION ( 'NONE',  ( -0.000000000000000000, -1.000000000000000000, -0.000000000000000000 ) ) ;
#29171=ORIENTED_EDGE ( 'NONE', *, *, #112319, .T. ) ;
#29172=FACE_BOUND ( 'NONE', #118081, .T. ) ;
#29173=EDGE_CURVE ( 'NONE', #31947, #104830, #36297, .T. ) ;
#29174=LINE ( 'NONE', #50727, #8144 ) ;
#29175=CARTESIAN_POINT ( 'NONE',  ( -11.89999999999999503, 12.50000000000000000, 4.048810130592458201 ) ) ;
#29176=EDGE_CURVE ( 'NONE', #27665, #108330, #63023, .T. ) ;
#29177=DIRECTION ( 'NONE',  ( -0.000000000000000000, -1.000000000000000000, -0.000000000000000000 ) ) ;
#29178=EDGE_CURVE ( 'NONE', #76002, #95427, #78501, .T. ) ;
#29180=FACE_OUTER_BOUND ( 'NONE', #64658, .T. ) ;
#29181=ADVANCED_FACE ( 'NONE', ( #115307 ), #83320, .T. ) ;
#29182=CARTESIAN_POINT ( 'NONE',  ( -3.100000000000028511, 2.500000000000000000, -4.676537180435977881 ) ) ;
#29183=EDGE_CURVE ( 'NONE', #95681, #18715, #84292, .T. ) ;
#29184=VERTEX_POINT ( 'NONE', #45974 ) ;
#29185=EDGE_CURVE ( 'NONE', #99172, #110598, #55049, .T. ) ;
#29186=AXIS2_PLACEMENT_3D ( 'NONE', #39548, #43397, #112774 ) ;
#29187=ORIENTED_EDGE ( 'NONE', *, *, #70254, .F. ) ;
#29188=VERTEX_POINT ( 'NONE', #74139 ) ;
#29189=ORIENTED_EDGE ( 'NONE', *, *, #102583, .F. ) ;
#29190=DIRECTION ( 'NONE',  ( 0.000000000000000000, 0.000000000000000000, -1.000000000000000000 ) ) ;
#29191=CARTESIAN_POINT ( 'NONE',  ( 4.599999999999936584, 2.500000000000000000, 4.330127018922196314 ) ) ;
#29192=CIRCLE ( 'NONE', #4023, 0.06509327318403745899 ) ;
#29193=EDGE_LOOP ( 'NONE', ( #21759, #1352, #6900, #10160 ) ) ;
#29194=ADVANCED_FACE ( 'NONE', ( #63679 ), #128229, .T. ) ;
#29195=CARTESIAN_POINT ( 'NONE',  ( 12.69999999999989981, 2.500000000000000000, -0.4464101615137783252 ) ) ;
#29196=EDGE_CURVE ( 'NONE', #66128, #15541, #96806, .T. ) ;
#29197=CARTESIAN_POINT ( 'NONE',  ( -15.59999999999998010, 12.50000000000000000, -0.3464101615137759604 ) ) ;
#29198=EDGE_CURVE ( 'NONE', #88710, #119959, #48806, .T. ) ;
#29199=CONICAL_SURFACE ( 'NONE', #81421, 0.1000000000000002554, 0.003490658503988666988 ) ;
#29200=FACE_OUTER_BOUND ( 'NONE', #81494, .T. ) ;
#29203=FACE_OUTER_BOUND ( 'NONE', #84235, .T. ) ;
#29204=DIRECTION ( 'NONE',  ( 0.000000000000000000, 1.000000000000000000, 0.000000000000000000 ) ) ;
#29205=AXIS2_PLACEMENT_3D ( 'NONE', #102414, #34334, #53320 ) ;
#29206=DIRECTION ( 'NONE',  ( 0.000000000000000000, 0.000000000000000000, 1.000000000000000000 ) ) ;
#29207=VERTEX_POINT ( 'NONE', #124532 ) ;
#29208=DIRECTION ( 'NONE',  ( 0.000000000000000000, 0.000000000000000000, 1.000000000000000000 ) ) ;
#29209=CIRCLE ( 'NONE', #66820, 0.09999999999999982514 ) ;
#29210=VERTEX_POINT ( 'NONE', #34875 ) ;
#29211=VERTEX_POINT ( 'NONE', #74782 ) ;
#29212=CARTESIAN_POINT ( 'NONE',  ( 8.149999999999923972, 2.500000000000000000, 2.511473670974873507 ) ) ;
#29213=CARTESIAN_POINT ( 'NONE',  ( -3.550000000000028244, 2.500000000000000000, 2.611473670974873151 ) ) ;
#29214=CARTESIAN_POINT ( 'NONE',  ( 1.849999999999950573, 2.500000000000000000, 2.511473670974873507 ) ) ;
#29215=ORIENTED_EDGE ( 'NONE', *, *, #72214, .F. ) ;
#29216=ORIENTED_EDGE ( 'NONE', *, *, #90518, .T. ) ;
#29217=CARTESIAN_POINT ( 'NONE',  ( 3.149999999999946176, 2.500000000000000000, -2.511473670974877948 ) ) ;
#29218=CARTESIAN_POINT ( 'NONE',  ( -0.8500000000000386136, 2.500000000000000000, 1.472243186433545459 ) ) ;
#29219=CARTESIAN_POINT ( 'NONE',  ( -3.100000000000028955, 2.500000000000000000, 4.576537180435972019 ) ) ;
#29220=CIRCLE ( 'NONE', #102368, 0.1000000000000002554 ) ;
#29221=ORIENTED_EDGE ( 'NONE', *, *, #90322, .T. ) ;
#29222=DIRECTION ( 'NONE',  ( -4.274815082592931898E-19, -0.9999939076577903929, -0.003490651415223739937 ) ) ;
#29223=VERTEX_POINT ( 'NONE', #64938 ) ;
#29224=FACE_OUTER_BOUND ( 'NONE', #105081, .T. ) ;
#29225=AXIS2_PLACEMENT_3D ( 'NONE', #20985, #91659, #41931 ) ;
#29226=AXIS2_PLACEMENT_3D ( 'NONE', #107138, #66569, #127446 ) ;
#29227=ORIENTED_EDGE ( 'NONE', *, *, #80000, .F. ) ;
#29228=DIRECTION ( 'NONE',  ( -0.000000000000000000, 1.000000000000000000, -0.000000000000000000 ) ) ;
#29229=DIRECTION ( 'NONE',  ( 0.000000000000000000, 1.000000000000000000, 0.000000000000000000 ) ) ;
#29230=CARTESIAN_POINT ( 'NONE',  ( -6.900000000000019007, 12.50000000000000000, -4.741630453620016006 ) ) ;
#29231=ADVANCED_FACE ( 'NONE', ( #24390 ), #63373, .T. ) ;
#29232=DIRECTION ( 'NONE',  ( 0.000000000000000000, 0.000000000000000000, 1.000000000000000000 ) ) ;
#29233=EDGE_LOOP ( 'NONE', ( #134, #7557, #77820, #31032 ) ) ;
#29234=AXIS2_PLACEMENT_3D ( 'NONE', #42268, #72378, #44183 ) ;
#29235=AXIS2_PLACEMENT_3D ( 'NONE', #27563, #45950, #125146 ) ;
#29236=ADVANCED_FACE ( 'NONE', ( #55140 ), #113541, .T. ) ;
#29237=DIRECTION ( 'NONE',  ( -0.000000000000000000, 1.000000000000000000, -0.000000000000000000 ) ) ;
#29238=EDGE_CURVE ( 'NONE', #84136, #107557, #78033, .T. ) ;
#29239=VERTEX_POINT ( 'NONE', #19051 ) ;
#29240=ORIENTED_EDGE ( 'NONE', *, *, #103566, .T. ) ;
#29241=CARTESIAN_POINT ( 'NONE',  ( 14.59999999999989484, 2.500000000000000000, -2.276824562219559311E-15 ) ) ;
#29242=CARTESIAN_POINT ( 'NONE',  ( 2.299999999999946976, 12.50000000000000000, 4.676537180435972552 ) ) ;
#29243=LINE ( 'NONE', #78988, #5151 ) ;
#29245=CARTESIAN_POINT ( 'NONE',  ( 9.999999999999912959, 2.500000000000000000, -5.022947341949754119 ) ) ;
#29246=EDGE_CURVE ( 'NONE', #69185, #12706, #46744, .T. ) ;
#29247=DIRECTION ( 'NONE',  ( -0.000000000000000000, 1.000000000000000000, -0.000000000000000000 ) ) ;
#29248=AXIS2_PLACEMENT_3D ( 'NONE', #114726, #5413, #25063 ) ;
#29249=CONICAL_SURFACE ( 'NONE', #102396, 0.1000000000000002554, 0.003490658503988666988 ) ;
#29250=DIRECTION ( 'NONE',  ( -0.000000000000000000, 1.000000000000000000, -0.000000000000000000 ) ) ;
#29251=DIRECTION ( 'NONE',  ( 0.000000000000000000, 0.000000000000000000, 1.000000000000000000 ) ) ;
#29252=CARTESIAN_POINT ( 'NONE',  ( 15.79999999999989058, 2.500000000000000000, 0.09999999999999761857 ) ) ;
#29253=CONICAL_SURFACE ( 'NONE', #66879, 0.1000000000000000056, 0.003490658503988666988 ) ;
#29254=EDGE_LOOP ( 'NONE', ( #54043, #101967 ) ) ;
#29255=VECTOR ( 'NONE', #74112, 1000.000000000000000 ) ;
#29257=DIRECTION ( 'NONE',  ( 0.000000000000000000, 0.000000000000000000, 1.000000000000000000 ) ) ;
#29258=LINE ( 'NONE', #15698, #78876 ) ;
#29259=EDGE_CURVE ( 'NONE', #74685, #66198, #25810, .T. ) ;
#29260=FACE_OUTER_BOUND ( 'NONE', #100562, .T. ) ;
#29261=CARTESIAN_POINT ( 'NONE',  ( 9.199999999999915801, 2.500000000000000000, 4.330127018922196314 ) ) ;
#29262=VERTEX_POINT ( 'NONE', #57053 ) ;
#29263=DIRECTION ( 'NONE',  ( -0.000000000000000000, -1.000000000000000000, -0.000000000000000000 ) ) ;
#29264=DIRECTION ( 'NONE',  ( -0.000000000000000000, 1.000000000000000000, -0.000000000000000000 ) ) ;
#29265=LINE ( 'NONE', #30566, #27518 ) ;
#29266=ORIENTED_EDGE ( 'NONE', *, *, #102136, .T. ) ;
#29267=VERTEX_POINT ( 'NONE', #57724 ) ;
#29268=DIRECTION ( 'NONE',  ( 0.000000000000000000, 0.000000000000000000, 1.000000000000000000 ) ) ;
#29269=EDGE_CURVE ( 'NONE', #85304, #103404, #66875, .T. ) ;
#29270=VERTEX_POINT ( 'NONE', #16475 ) ;
#29271=VERTEX_POINT ( 'NONE', #128413 ) ;
#29272=EDGE_LOOP ( 'NONE', ( #7401, #47047 ) ) ;
#29273=DIRECTION ( 'NONE',  ( 0.000000000000000000, 0.000000000000000000, 1.000000000000000000 ) ) ;
#29274=CONICAL_SURFACE ( 'NONE', #102430, 0.1000000000000000056, 0.003490658503988666988 ) ;
#29275=CARTESIAN_POINT ( 'NONE',  ( 3.349999999999942801, 12.50000000000000000, 2.857883832488649301 ) ) ;
#29276=FACE_OUTER_BOUND ( 'NONE', #67210, .T. ) ;
#29277=CARTESIAN_POINT ( 'NONE',  ( 2.949999999999946887, 2.500000000000000000, -6.595190528383302109 ) ) ;
#29278=EDGE_LOOP ( 'NONE', ( #116737, #23005 ) ) ;
#29279=CONICAL_SURFACE ( 'NONE', #56446, 0.09999999999999982514, 0.003490658503988666988 ) ;
#29280=DIRECTION ( 'NONE',  ( 0.000000000000000000, 1.000000000000000000, 0.000000000000000000 ) ) ;
#29281=ORIENTED_EDGE ( 'NONE', *, *, #61721, .T. ) ;
#29282=DIRECTION ( 'NONE',  ( 0.000000000000000000, 0.000000000000000000, 1.000000000000000000 ) ) ;
#29283=CARTESIAN_POINT ( 'NONE',  ( 16.86689433361522461, 2.548103353434407747, 5.776876940644654290 ) ) ;
#29284=CARTESIAN_POINT ( 'NONE',  ( 6.649999999999927525, 2.500000000000000000, 2.065063509461097624 ) ) ;
#29285=ADVANCED_FACE ( 'NONE', ( #66232 ), #56414, .T. ) ;
#29286=DIRECTION ( 'NONE',  ( 0.000000000000000000, 0.000000000000000000, -1.000000000000000000 ) ) ;
#29287=ORIENTED_EDGE ( 'NONE', *, *, #60916, .T. ) ;
#29288=AXIS2_PLACEMENT_3D ( 'NONE', #127136, #106199, #56434 ) ;
#29289=AXIS2_PLACEMENT_3D ( 'NONE', #7855, #7204, #6531 ) ;
#29290=ORIENTED_EDGE ( 'NONE', *, *, #57717, .T. ) ;
#29291=ORIENTED_EDGE ( 'NONE', *, *, #115934, .F. ) ;
#29292=VERTEX_POINT ( 'NONE', #127110 ) ;
#29293=ORIENTED_EDGE ( 'NONE', *, *, #4601, .T. ) ;
#29294=CARTESIAN_POINT ( 'NONE',  ( -5.400000000000023448, 12.50000000000000000, -4.330127018922201643 ) ) ;
#29295=DIRECTION ( 'NONE',  ( 0.000000000000000000, -0.9999939076577903929, 0.003490651415223739937 ) ) ;
#29296=EDGE_CURVE ( 'NONE', #58654, #12633, #96329, .T. ) ;
#29297=DIRECTION ( 'NONE',  ( -4.274815082592931898E-19, -0.9999939076577903929, -0.003490651415223739937 ) ) ;
#29298=FACE_BOUND ( 'NONE', #76187, .T. ) ;
#29299=DIRECTION ( 'NONE',  ( 0.000000000000000000, 1.000000000000000000, 0.000000000000000000 ) ) ;
#29301=DIRECTION ( 'NONE',  ( 0.000000000000000000, -0.000000000000000000, 1.000000000000000000 ) ) ;
#29302=FACE_OUTER_BOUND ( 'NONE', #87189, .T. ) ;
#29303=DIRECTION ( 'NONE',  ( 0.000000000000000000, 0.000000000000000000, 1.000000000000000000 ) ) ;
#29305=DIRECTION ( 'NONE',  ( 0.000000000000000000, -0.9999939076577903929, 0.003490651415223739937 ) ) ;
#29306=CONICAL_SURFACE ( 'NONE', #31457, 0.09999999999999999167, 0.003490658503988666988 ) ;
#29307=DIRECTION ( 'NONE',  ( 0.000000000000000000, 1.000000000000000000, 0.000000000000000000 ) ) ;
#29308=EDGE_CURVE ( 'NONE', #76747, #104576, #27861, .T. ) ;
#29309=ORIENTED_EDGE ( 'NONE', *, *, #47576, .F. ) ;
#29310=ORIENTED_EDGE ( 'NONE', *, *, #54545, .F. ) ;
#29311=ORIENTED_EDGE ( 'NONE', *, *, #57561, .F. ) ;
#29312=ORIENTED_EDGE ( 'NONE', *, *, #43933, .T. ) ;
#29313=CARTESIAN_POINT ( 'NONE',  ( -12.09999999999999609, 2.500000000000000000, 0.7928203230275536750 ) ) ;
#29314=CARTESIAN_POINT ( 'NONE',  ( 0.5999999999999555689, 2.500000000000000000, 4.576537180435972019 ) ) ;
#29315=FACE_BOUND ( 'NONE', #96771, .T. ) ;
#29316=CIRCLE ( 'NONE', #27242, 0.06509327318403741736 ) ;
#29317=DIRECTION ( 'NONE',  ( 0.000000000000000000, 0.000000000000000000, 1.000000000000000000 ) ) ;
#29318=ADVANCED_FACE ( 'NONE', ( #67506 ), #65504, .T. ) ;
#29319=EDGE_LOOP ( 'NONE', ( #21798, #61844 ) ) ;
#29320=EDGE_CURVE ( 'NONE', #105793, #15536, #40400, .T. ) ;
#29321=PLANE ( 'NONE',  #75955 ) ;
#29322=CARTESIAN_POINT ( 'NONE',  ( -11.25000000000000000, 2.500000000000000000, 2.757883832488649656 ) ) ;
#29323=ADVANCED_FACE ( 'NONE', ( #86518 ), #119893, .T. ) ;
#29324=DIRECTION ( 'NONE',  ( 0.000000000000000000, -0.9999939076577903929, 0.003490651415223739937 ) ) ;
#29325=FACE_OUTER_BOUND ( 'NONE', #73135, .T. ) ;
#29326=ADVANCED_FACE ( 'NONE', ( #7957 ), #15323, .T. ) ;
#29327=CARTESIAN_POINT ( 'NONE',  ( 7.099999999999928590, 12.50000000000000000, -4.330127018922201643 ) ) ;
#29328=AXIS2_PLACEMENT_3D ( 'NONE', #16390, #85794, #65513 ) ;
#29329=EDGE_CURVE ( 'NONE', #7687, #50249, #116622, .T. ) ;
#29331=CARTESIAN_POINT ( 'NONE',  ( 4.599999999999940137, 2.500000000000000000, -5.022947341949754119 ) ) ;
#29332=VECTOR ( 'NONE', #93017, 1000.000000000000000 ) ;
#29333=AXIS2_PLACEMENT_3D ( 'NONE', #122979, #119, #89160 ) ;
#29334=ORIENTED_EDGE ( 'NONE', *, *, #17755, .F. ) ;
#29335=EDGE_CURVE ( 'NONE', #22598, #116333, #98963, .T. ) ;
#29336=EDGE_LOOP ( 'NONE', ( #21621, #99236 ) ) ;
#29337=CARTESIAN_POINT ( 'NONE',  ( 6.649999999999930189, 12.50000000000000000, 7.122917578226811486 ) ) ;
#29338=ADVANCED_FACE ( 'NONE', ( #129055 ), #111482, .T. ) ;
#29339=CARTESIAN_POINT ( 'NONE',  ( -0.4000000000000331624, 12.50000000000000000, 0.000000000000000000 ) ) ;
#29340=ORIENTED_EDGE ( 'NONE', *, *, #120908, .F. ) ;
#29341=EDGE_CURVE ( 'NONE', #33171, #56826, #32083, .T. ) ;
#29342=CIRCLE ( 'NONE', #96206, 0.06509327318403745899 ) ;
#29343=ADVANCED_FACE ( 'NONE', ( #118556 ), #105221, .T. ) ;
#29344=CARTESIAN_POINT ( 'NONE',  ( 8.349999999999919709, 2.500000000000000000, 6.595190528383296780 ) ) ;
#29345=EDGE_CURVE ( 'NONE', #93190, #43830, #9259, .T. ) ;
#29346=DIRECTION ( 'NONE',  ( -0.000000000000000000, -1.000000000000000000, -0.000000000000000000 ) ) ;
#29347=EDGE_LOOP ( 'NONE', ( #55017, #84769, #78861, #82899 ) ) ;
#29348=CARTESIAN_POINT ( 'NONE',  ( 2.049999999999948308, 12.50000000000000000, 6.495190528383297135 ) ) ;
#29349=AXIS2_PLACEMENT_3D ( 'NONE', #98191, #37357, #7216 ) ;
#29350=VERTEX_POINT ( 'NONE', #99584 ) ;
#29351=DIRECTION ( 'NONE',  ( 0.000000000000000000, 0.000000000000000000, 1.000000000000000000 ) ) ;
#29352=ADVANCED_FACE ( 'NONE', ( #1358 ), #86432, .T. ) ;
#29353=EDGE_LOOP ( 'NONE', ( #48852, #103251 ) ) ;
#29354=CARTESIAN_POINT ( 'NONE',  ( 5.849999999999935696, 2.500000000000000000, -7.188010851410854052 ) ) ;
#29355=FACE_BOUND ( 'NONE', #107959, .T. ) ;
#29356=ORIENTED_EDGE ( 'NONE', *, *, #116485, .F. ) ;
#29357=CARTESIAN_POINT ( 'NONE',  ( -5.400000000000020783, 2.500000000000000000, 0.6928203230275494784 ) ) ;
#29358=ORIENTED_EDGE ( 'NONE', *, *, #50456, .F. ) ;
#29360=LINE ( 'NONE', #60742, #105212 ) ;
#29363=CARTESIAN_POINT ( 'NONE',  ( -4.600000000000024514, 12.50000000000000000, 5.022947341949748790 ) ) ;
#29364=ORIENTED_EDGE ( 'NONE', *, *, #87253, .T. ) ;
#29365=ORIENTED_EDGE ( 'NONE', *, *, #94325, .T. ) ;
#29366=VERTEX_POINT ( 'NONE', #111296 ) ;
#29367=FACE_OUTER_BOUND ( 'NONE', #75407, .T. ) ;
#29368=FACE_OUTER_BOUND ( 'NONE', #82699, .T. ) ;
#29369=AXIS2_PLACEMENT_3D ( 'NONE', #32459, #80893, #90703 ) ;
#29370=DIRECTION ( 'NONE',  ( 0.000000000000000000, 1.000000000000000000, 0.000000000000000000 ) ) ;
#29371=EDGE_LOOP ( 'NONE', ( #83777, #14926 ) ) ;
#29372=ORIENTED_EDGE ( 'NONE', *, *, #58574, .F. ) ;
#29373=ORIENTED_EDGE ( 'NONE', *, *, #54256, .F. ) ;
#29374=CONICAL_SURFACE ( 'NONE', #10556, 0.1000000000000002554, 0.003490658503988666988 ) ;
#29375=DIRECTION ( 'NONE',  ( -0.000000000000000000, -1.000000000000000000, -0.000000000000000000 ) ) ;
#29376=DIRECTION ( 'NONE',  ( 0.000000000000000000, 0.000000000000000000, 1.000000000000000000 ) ) ;
#29378=CONICAL_SURFACE ( 'NONE', #25148, 0.09999999999999982514, 0.003490658503988666988 ) ;
#29379=VECTOR ( 'NONE', #94478, 1000.000000000000000 ) ;
#29380=DIRECTION ( 'NONE',  ( 0.000000000000000000, 0.000000000000000000, -1.000000000000000000 ) ) ;
#29381=DIRECTION ( 'NONE',  ( 0.000000000000000000, 1.000000000000000000, 0.000000000000000000 ) ) ;
#29382=FACE_OUTER_BOUND ( 'NONE', #62896, .T. ) ;
#29383=CARTESIAN_POINT ( 'NONE',  ( -10.84999999999999964, 12.50000000000000000, 7.122917578226811486 ) ) ;
#29384=DIRECTION ( 'NONE',  ( 0.000000000000000000, 1.000000000000000000, 0.000000000000000000 ) ) ;
#29385=CARTESIAN_POINT ( 'NONE',  ( 13.34999999999989662, 2.500000000000000000, -2.757883832488654097 ) ) ;
#29386=EDGE_LOOP ( 'NONE', ( #94260, #106507, #19217, #22736 ) ) ;
#29387=ORIENTED_EDGE ( 'NONE', *, *, #58998, .T. ) ;
#29388=EDGE_CURVE ( 'NONE', #19644, #103729, #21661, .T. ) ;
#29389=DIRECTION ( 'NONE',  ( -0.000000000000000000, 1.000000000000000000, -0.000000000000000000 ) ) ;
#29390=EDGE_CURVE ( 'NONE', #84227, #69984, #41953, .T. ) ;
#29391=CARTESIAN_POINT ( 'NONE',  ( 6.049999999999932321, 12.50000000000000000, 6.841600689897072485 ) ) ;
#29392=EDGE_LOOP ( 'NONE', ( #62358, #74356 ) ) ;
#29393=ORIENTED_EDGE ( 'NONE', *, *, #24321, .T. ) ;
#29395=FACE_OUTER_BOUND ( 'NONE', #61343, .T. ) ;
#29396=CARTESIAN_POINT ( 'NONE',  ( 8.749999999999953815, 12.50000000000000000, -2.099970236277064473 ) ) ;
#29397=EDGE_CURVE ( 'NONE', #46240, #48600, #9901, .T. ) ;
#29398=DIRECTION ( 'NONE',  ( 0.000000000000000000, 0.000000000000000000, 1.000000000000000000 ) ) ;
#29399=CARTESIAN_POINT ( 'NONE',  ( 12.04999999999990479, 2.500000000000000000, 2.165063509461097713 ) ) ;
#29400=CARTESIAN_POINT ( 'NONE',  ( -6.050000000000020250, 2.500000000000000000, -6.841600689897078702 ) ) ;
#29401=CARTESIAN_POINT ( 'NONE',  ( -13.09999999999999254, 12.50000000000000000, -4.676537180435975216 ) ) ;
#29402=CARTESIAN_POINT ( 'NONE',  ( 0.8499999999999545697, 12.50000000000000000, -1.472243186433550122 ) ) ;
#29403=VECTOR ( 'NONE', #41328, 1000.000000000000000 ) ;
#29404=CIRCLE ( 'NONE', #27313, 0.06509327318403745899 ) ;
#29405=EDGE_LOOP ( 'NONE', ( #39247, #85397, #60714, #126785 ) ) ;
#29406=ORIENTED_EDGE ( 'NONE', *, *, #10123, .F. ) ;
#29407=EDGE_LOOP ( 'NONE', ( #73400, #128312 ) ) ;
#29408=ORIENTED_EDGE ( 'NONE', *, *, #36845, .T. ) ;
#29409=DIRECTION ( 'NONE',  ( -0.000000000000000000, -1.000000000000000000, -0.000000000000000000 ) ) ;
#29410=CARTESIAN_POINT ( 'NONE',  ( -3.150000000000033218, 2.500000000000000000, -6.841600689897078702 ) ) ;
#29411=CONICAL_SURFACE ( 'NONE', #48183, 0.1000000000000002554, 0.003490658503988666988 ) ;
#29412=VERTEX_POINT ( 'NONE', #121140 ) ;
#29413=CARTESIAN_POINT ( 'NONE',  ( 9.349999999999919709, 2.500000000000000000, 1.718653347947321386 ) ) ;
#29414=CARTESIAN_POINT ( 'NONE',  ( 3.749999999999978684, 2.500000000000000000, -2.165063509461101710 ) ) ;
#29415=DIRECTION ( 'NONE',  ( 0.000000000000000000, 0.000000000000000000, 1.000000000000000000 ) ) ;
#29416=CARTESIAN_POINT ( 'NONE',  ( 0.7999999999999612976, 12.50000000000000000, -1.084202172485504434E-16 ) ) ;
#29417=ORIENTED_EDGE ( 'NONE', *, *, #42037, .T. ) ;
#29418=DIRECTION ( 'NONE',  ( -0.000000000000000000, -1.000000000000000000, -0.000000000000000000 ) ) ;
#29419=FACE_OUTER_BOUND ( 'NONE', #96747, .T. ) ;
#29420=AXIS2_PLACEMENT_3D ( 'NONE', #49082, #58251, #59561 ) ;
#29421=ADVANCED_FACE ( 'NONE', ( #20370 ), #62238, .T. ) ;
#29422=EDGE_LOOP ( 'NONE', ( #106292, #53386, #103981, #42420 ) ) ;
#29423=VECTOR ( 'NONE', #39137, 1000.000000000000000 ) ;
#29425=ORIENTED_EDGE ( 'NONE', *, *, #108634, .F. ) ;
#29427=DIRECTION ( 'NONE',  ( 0.000000000000000000, -0.000000000000000000, 1.000000000000000000 ) ) ;
#29428=CIRCLE ( 'NONE', #31570, 0.09999999999999982514 ) ;
#29429=CARTESIAN_POINT ( 'NONE',  ( 11.04999999999990834, 12.50000000000000000, -6.776507416713039689 ) ) ;
#29430=CARTESIAN_POINT ( 'NONE',  ( -5.850000000000019185, 12.50000000000000000, 6.495190528383297135 ) ) ;
#29431=AXIS2_PLACEMENT_3D ( 'NONE', #35742, #105771, #106406 ) ;
#29432=EDGE_CURVE ( 'NONE', #60192, #13704, #7094, .T. ) ;
#29433=EDGE_LOOP ( 'NONE', ( #51187, #112939, #68812, #24899 ) ) ;
#29434=DIRECTION ( 'NONE',  ( 0.000000000000000000, 0.000000000000000000, -1.000000000000000000 ) ) ;
#29435=FACE_OUTER_BOUND ( 'NONE', #22637, .T. ) ;
#29436=DIRECTION ( 'NONE',  ( 0.000000000000000000, -0.000000000000000000, 1.000000000000000000 ) ) ;
#29437=LINE ( 'NONE', #40564, #31734 ) ;
#29438=ADVANCED_FACE ( 'NONE', ( #39392 ), #40678, .T. ) ;
#29439=ORIENTED_EDGE ( 'NONE', *, *, #75564, .F. ) ;
#29441=ORIENTED_EDGE ( 'NONE', *, *, #18647, .T. ) ;
#29442=VERTEX_POINT ( 'NONE', #121773 ) ;
#29443=FACE_OUTER_BOUND ( 'NONE', #113295, .T. ) ;
#29444=EDGE_CURVE ( 'NONE', #40822, #100700, #119211, .T. ) ;
#29445=DIRECTION ( 'NONE',  ( 0.000000000000000000, 0.000000000000000000, 1.000000000000000000 ) ) ;
#29446=FACE_BOUND ( 'NONE', #78400, .T. ) ;
#29447=DIRECTION ( 'NONE',  ( 0.000000000000000000, 0.000000000000000000, -1.000000000000000000 ) ) ;
#29449=DIRECTION ( 'NONE',  ( 0.000000000000000000, -0.9999939076577903929, 0.003490651415223739937 ) ) ;
#29450=CIRCLE ( 'NONE', #35707, 0.06509327318403745899 ) ;
#29451=AXIS2_PLACEMENT_3D ( 'NONE', #80751, #71556, #70922 ) ;
#29452=EDGE_LOOP ( 'NONE', ( #52049, #70215 ) ) ;
#29453=FACE_OUTER_BOUND ( 'NONE', #37536, .T. ) ;
#29455=DIRECTION ( 'NONE',  ( -0.000000000000000000, 1.000000000000000000, -0.000000000000000000 ) ) ;
#29456=LINE ( 'NONE', #110582, #13109 ) ;
#29458=EDGE_LOOP ( 'NONE', ( #60417, #81177 ) ) ;
#29459=DIRECTION ( 'NONE',  ( 0.000000000000000000, 0.000000000000000000, 1.000000000000000000 ) ) ;
#29460=CIRCLE ( 'NONE', #73357, 0.06509327318403743123 ) ;
#29461=CARTESIAN_POINT ( 'NONE',  ( 8.949999999999917577, 2.500000000000000000, 6.148780366869520009 ) ) ;
#29462=ORIENTED_EDGE ( 'NONE', *, *, #52511, .T. ) ;
#29463=VERTEX_POINT ( 'NONE', #49842 ) ;
#29464=PLANE ( 'NONE',  #100357 ) ;
#29465=CARTESIAN_POINT ( 'NONE',  ( 14.34999999999989306, 2.500000000000000000, -2.511473670974877948 ) ) ;
#29466=FACE_BOUND ( 'NONE', #755, .T. ) ;
#29467=CARTESIAN_POINT ( 'NONE',  ( 2.299999999999949640, 2.500000000000000000, -0.3464101615137782364 ) ) ;
#29468=EDGE_CURVE ( 'NONE', #53781, #56111, #25899, .T. ) ;
#29469=CARTESIAN_POINT ( 'NONE',  ( 4.999999999999935163, 2.500000000000000000, 3.637306695894644726 ) ) ;
#29470=ORIENTED_EDGE ( 'NONE', *, *, #4632, .T. ) ;
#29471=FACE_OUTER_BOUND ( 'NONE', #76076, .T. ) ;
#29472=EDGE_CURVE ( 'NONE', #70518, #42007, #27952, .T. ) ;
#29474=EDGE_CURVE ( 'NONE', #2432, #29267, #124092, .T. ) ;
#29475=ORIENTED_EDGE ( 'NONE', *, *, #83564, .T. ) ;
#29476=DIRECTION ( 'NONE',  ( -4.274815082592931898E-19, -0.9999939076577903929, -0.003490651415223739937 ) ) ;
#29477=CARTESIAN_POINT ( 'NONE',  ( 1.899999999999949507, 12.50000000000000000, 4.676537180435972552 ) ) ;
#29478=VECTOR ( 'NONE', #58808, 1000.000000000000000 ) ;
#29479=EDGE_CURVE ( 'NONE', #64667, #32289, #34239, .T. ) ;
#29480=ADVANCED_FACE ( 'NONE', ( #81846 ), #101510, .T. ) ;
#29481=CARTESIAN_POINT ( 'NONE',  ( 6.649999999999931966, 12.50000000000000000, -5.802370205355749988 ) ) ;
#29482=EDGE_CURVE ( 'NONE', #105720, #95522, #70118, .T. ) ;
#29483=DIRECTION ( 'NONE',  ( 0.000000000000000000, -0.9999939076577903929, 0.003490651415223739937 ) ) ;
#29484=AXIS2_PLACEMENT_3D ( 'NONE', #63180, #122744, #44176 ) ;
#29485=ORIENTED_EDGE ( 'NONE', *, *, #89886, .T. ) ;
#29487=EDGE_CURVE ( 'NONE', #63009, #105656, #119996, .T. ) ;
#29488=CARTESIAN_POINT ( 'NONE',  ( -9.999999999999969802, 2.500000000000000000, -2.276824562219559311E-15 ) ) ;
#29489=DIRECTION ( 'NONE',  ( -4.274815082592931898E-19, -0.9999939076577903929, -0.003490651415223739937 ) ) ;
#29490=CARTESIAN_POINT ( 'NONE',  ( 11.44999999999991047, 2.500000000000000000, -2.511473670974877948 ) ) ;
#29492=ORIENTED_EDGE ( 'NONE', *, *, #64625, .F. ) ;
#29493=CARTESIAN_POINT ( 'NONE',  ( -13.54999999999998828, 2.500000000000000000, -2.511473670974875727 ) ) ;
#29494=VECTOR ( 'NONE', #34757, 1000.000000000000000 ) ;
#29495=ADVANCED_FACE ( 'NONE', ( #70754 ), #7000, .T. ) ;
#29496=ORIENTED_EDGE ( 'NONE', *, *, #88736, .F. ) ;
#29497=CARTESIAN_POINT ( 'NONE',  ( -11.64999999999999680, 2.500000000000000000, 7.088010851410848190 ) ) ;
#29498=CIRCLE ( 'NONE', #50415, 0.06509327318403745899 ) ;
#29499=CARTESIAN_POINT ( 'NONE',  ( 17.50000000000000000, -2.499999999999999556, 3.666666666666668739 ) ) ;
#29500=CARTESIAN_POINT ( 'NONE',  ( 11.04999999999990834, 2.500000000000000000, -6.841600689897077814 ) ) ;
#29501=ORIENTED_EDGE ( 'NONE', *, *, #116820, .T. ) ;
#29502=CARTESIAN_POINT ( 'NONE',  ( 4.199999999999939782, 12.50000000000000000, -2.276824562219559311E-15 ) ) ;
#29503=FACE_OUTER_BOUND ( 'NONE', #104371, .T. ) ;
#29504=CARTESIAN_POINT ( 'NONE',  ( -5.400000000000020783, 12.50000000000000000, 0.7579135962115869374 ) ) ;
#29505=LINE ( 'NONE', #9863, #39102 ) ;
#29506=DIRECTION ( 'NONE',  ( 0.000000000000000000, 0.000000000000000000, 1.000000000000000000 ) ) ;
#29507=DIRECTION ( 'NONE',  ( 0.000000000000000000, 1.000000000000000000, 0.000000000000000000 ) ) ;
#29508=CIRCLE ( 'NONE', #8638, 0.1000000000000002554 ) ;
#29509=ORIENTED_EDGE ( 'NONE', *, *, #11719, .F. ) ;
#29510=AXIS2_PLACEMENT_3D ( 'NONE', #10896, #50860, #101892 ) ;
#29511=EDGE_LOOP ( 'NONE', ( #71415, #94151, #61794, #22815 ) ) ;
#29512=DIRECTION ( 'NONE',  ( -0.000000000000000000, 1.000000000000000000, -0.000000000000000000 ) ) ;
#29513=VERTEX_POINT ( 'NONE', #22321 ) ;
#29515=ORIENTED_EDGE ( 'NONE', *, *, #29432, .T. ) ;
#29516=EDGE_LOOP ( 'NONE', ( #119860, #75810, #33518, #78928 ) ) ;
#29517=EDGE_LOOP ( 'NONE', ( #113054, #41607 ) ) ;
#29518=PLANE ( 'NONE',  #73040 ) ;
#29519=CIRCLE ( 'NONE', #125640, 0.1000000000000000472 ) ;
#29520=CARTESIAN_POINT ( 'NONE',  ( 11.24999999999994316, 2.500000000000000000, 2.065063509461097624 ) ) ;
#29521=CARTESIAN_POINT ( 'NONE',  ( -5.400000000000020783, 2.500000000000000000, 4.922947341949748257 ) ) ;
#29523=CARTESIAN_POINT ( 'NONE',  ( 11.04999999999990834, 12.50000000000000000, -6.841600689897077814 ) ) ;
#29524=AXIS2_PLACEMENT_3D ( 'NONE', #97874, #70355, #60562 ) ;
#29525=VECTOR ( 'NONE', #75092, 1000.000000000000000 ) ;
#29526=DIRECTION ( 'NONE',  ( -0.000000000000000000, 1.000000000000000000, -0.000000000000000000 ) ) ;
#29527=DIRECTION ( 'NONE',  ( 0.000000000000000000, 0.000000000000000000, 1.000000000000000000 ) ) ;
#29528=CARTESIAN_POINT ( 'NONE',  ( 6.849999999999927702, 2.500000000000000000, 1.818653347947321475 ) ) ;
#29529=CARTESIAN_POINT ( 'NONE',  ( 13.29999999999990301, 2.500000000000000000, 4.430127018922196847 ) ) ;
#29530=DIRECTION ( 'NONE',  ( -0.000000000000000000, 1.000000000000000000, -0.000000000000000000 ) ) ;
#29531=EDGE_LOOP ( 'NONE', ( #128637, #120270 ) ) ;
#29532=EDGE_LOOP ( 'NONE', ( #62621, #23387, #66843, #76365 ) ) ;
#29533=EDGE_CURVE ( 'NONE', #62131, #43475, #2923, .T. ) ;
#29534=DIRECTION ( 'NONE',  ( 0.000000000000000000, 0.000000000000000000, 1.000000000000000000 ) ) ;
#29535=ORIENTED_EDGE ( 'NONE', *, *, #18790, .F. ) ;
#29536=ORIENTED_EDGE ( 'NONE', *, *, #41169, .F. ) ;
#29537=CARTESIAN_POINT ( 'NONE',  ( 7.499999999999925393, 2.500000000000000000, -0.5928203230275541635 ) ) ;
#29538=ADVANCED_FACE ( 'NONE', ( #73978 ), #128321, .T. ) ;
#29539=CARTESIAN_POINT ( 'NONE',  ( -7.700000000000016165, 2.500000000000000000, -4.083716857408426826 ) ) ;
#29540=DIRECTION ( 'NONE',  ( -4.274815082592931898E-19, -0.9999939076577903929, -0.003490651415223739937 ) ) ;
#29541=CONICAL_SURFACE ( 'NONE', #10725, 0.1000000000000000472, 0.003490658503988666988 ) ;
#29542=CARTESIAN_POINT ( 'NONE',  ( 9.999999999999916511, 12.50000000000000000, -0.6928203230275541413 ) ) ;
#29543=ORIENTED_EDGE ( 'NONE', *, *, #108190, .T. ) ;
#29544=AXIS2_PLACEMENT_3D ( 'NONE', #108742, #118564, #89113 ) ;
#29545=CIRCLE ( 'NONE', #10726, 0.1000000000000000472 ) ;
#29546=ORIENTED_EDGE ( 'NONE', *, *, #107956, .T. ) ;
#29547=DIRECTION ( 'NONE',  ( 0.000000000000000000, 0.000000000000000000, -1.000000000000000000 ) ) ;
#29548=VERTEX_POINT ( 'NONE', #32789 ) ;
#29549=DIRECTION ( 'NONE',  ( 0.000000000000000000, 0.000000000000000000, -1.000000000000000000 ) ) ;
#29550=ORIENTED_EDGE ( 'NONE', *, *, #94428, .T. ) ;
#29551=CIRCLE ( 'NONE', #108945, 0.06509327318403745899 ) ;
#29552=ORIENTED_EDGE ( 'NONE', *, *, #70162, .F. ) ;
#29553=DIRECTION ( 'NONE',  ( 0.000000000000000000, 0.000000000000000000, -1.000000000000000000 ) ) ;
#29554=CARTESIAN_POINT ( 'NONE',  ( 81.97061111377811926, -3.937853021331575221, -6.123961096638185886 ) ) ;
#29555=DIRECTION ( 'NONE',  ( 0.000000000000000000, -0.9999939076577903929, 0.003490651415223739937 ) ) ;
#29556=DIRECTION ( 'NONE',  ( 0.000000000000000000, -0.000000000000000000, 1.000000000000000000 ) ) ;
#29557=CARTESIAN_POINT ( 'NONE',  ( 0.8499999999999536815, 12.50000000000000000, 6.430097255199259010 ) ) ;
#29558=ORIENTED_EDGE ( 'NONE', *, *, #121927, .F. ) ;
#29559=DIRECTION ( 'NONE',  ( 0.000000000000000000, 0.000000000000000000, 1.000000000000000000 ) ) ;
#29560=FACE_OUTER_BOUND ( 'NONE', #4705, .T. ) ;
#29561=DIRECTION ( 'NONE',  ( 0.000000000000000000, 0.000000000000000000, 1.000000000000000000 ) ) ;
#29562=DIRECTION ( 'NONE',  ( 0.000000000000000000, 0.000000000000000000, -1.000000000000000000 ) ) ;
#29563=CARTESIAN_POINT ( 'NONE',  ( -8.950000000000006395, 2.500000000000000000, 6.841600689897072485 ) ) ;
#29564=ADVANCED_FACE ( 'NONE', ( #55622 ), #24234, .T. ) ;
#29565=EDGE_LOOP ( 'NONE', ( #115627, #73761, #80403, #23448 ) ) ;
#29566=EDGE_LOOP ( 'NONE', ( #12908, #87989 ) ) ;
#29567=DIRECTION ( 'NONE',  ( -4.274815082592931898E-19, -0.9999939076577903929, -0.003490651415223739937 ) ) ;
#29568=ORIENTED_EDGE ( 'NONE', *, *, #14711, .F. ) ;
#29569=CARTESIAN_POINT ( 'NONE',  ( 17.48308156489508747, -2.102418598455126020, 4.293689242909404236 ) ) ;
#29570=AXIS2_PLACEMENT_3D ( 'NONE', #12957, #73191, #24094 ) ;
#29571=DIRECTION ( 'NONE',  ( -4.274815082592931898E-19, -0.9999939076577903929, -0.003490651415223739937 ) ) ;
#29572=EDGE_CURVE ( 'NONE', #88750, #30265, #54971, .T. ) ;
#29573=EDGE_CURVE ( 'NONE', #32088, #7687, #80194, .T. ) ;
#29574=ORIENTED_EDGE ( 'NONE', *, *, #126983, .F. ) ;
#29575=LINE ( 'NONE', #111336, #57840 ) ;
#29576=DIRECTION ( 'NONE',  ( 0.000000000000000000, 0.000000000000000000, 1.000000000000000000 ) ) ;
#29577=DIRECTION ( 'NONE',  ( 0.000000000000000000, 1.000000000000000000, 0.000000000000000000 ) ) ;
#29578=ADVANCED_FACE ( 'NONE', ( #2636 ), #63557, .T. ) ;
#29579=DIRECTION ( 'NONE',  ( 0.000000000000000000, -0.9999939076577903929, 0.003490651415223739937 ) ) ;
#29580=AXIS2_PLACEMENT_3D ( 'NONE', #92205, #2525, #122338 ) ;
#29581=AXIS2_PLACEMENT_3D ( 'NONE', #48379, #50315, #18903 ) ;
#29582=DIRECTION ( 'NONE',  ( 0.000000000000000000, 0.000000000000000000, 1.000000000000000000 ) ) ;
#29583=EDGE_CURVE ( 'NONE', #86749, #32777, #22950, .T. ) ;
#29584=VERTEX_POINT ( 'NONE', #82525 ) ;
#29585=ADVANCED_FACE ( 'NONE', ( #122441 ), #44689, .T. ) ;
#29586=DIRECTION ( 'NONE',  ( 0.000000000000000000, -0.000000000000000000, 1.000000000000000000 ) ) ;
#29587=DIRECTION ( 'NONE',  ( 0.000000000000000000, 0.000000000000000000, 1.000000000000000000 ) ) ;
#29588=CARTESIAN_POINT ( 'NONE',  ( -4.294665249841745289E-14, 2.500000000000000000, 4.922947341949748257 ) ) ;
#29589=CIRCLE ( 'NONE', #108994, 0.06509327318403745899 ) ;
#29590=CIRCLE ( 'NONE', #14888, 0.1000000000000002554 ) ;
#29591=ORIENTED_EDGE ( 'NONE', *, *, #3601, .F. ) ;
#29592=DIRECTION ( 'NONE',  ( 0.000000000000000000, 0.000000000000000000, 1.000000000000000000 ) ) ;
#29593=AXIS2_PLACEMENT_3D ( 'NONE', #111685, #10869, #50828 ) ;
#29594=ORIENTED_EDGE ( 'NONE', *, *, #123882, .T. ) ;
#29595=DIRECTION ( 'NONE',  ( 0.000000000000000000, -0.9999939076577903929, 0.003490651415223739937 ) ) ;
#29596=PLANE ( 'NONE',  #119815 ) ;
#29597=VECTOR ( 'NONE', #89341, 1000.000000000000000 ) ;
#29598=DIRECTION ( 'NONE',  ( 0.000000000000000000, 1.000000000000000000, 0.000000000000000000 ) ) ;
#29599=ORIENTED_EDGE ( 'NONE', *, *, #120436, .F. ) ;
#29600=DIRECTION ( 'NONE',  ( 0.000000000000000000, 1.000000000000000000, 0.000000000000000000 ) ) ;
#29601=DIRECTION ( 'NONE',  ( -0.000000000000000000, 1.000000000000000000, -0.000000000000000000 ) ) ;
#29602=CIRCLE ( 'NONE', #77620, 0.06509327318403745899 ) ;
#29603=VECTOR ( 'NONE', #103104, 1000.000000000000000 ) ;
#29604=ORIENTED_EDGE ( 'NONE', *, *, #58155, .T. ) ;
#29605=DIRECTION ( 'NONE',  ( 0.000000000000000000, 0.000000000000000000, 1.000000000000000000 ) ) ;
#29606=ORIENTED_EDGE ( 'NONE', *, *, #59743, .F. ) ;
#29607=DIRECTION ( 'NONE',  ( 0.000000000000000000, 0.000000000000000000, 1.000000000000000000 ) ) ;
#29608=ADVANCED_FACE ( 'NONE', ( #13099 ), #48900, .T. ) ;
#29609=EDGE_LOOP ( 'NONE', ( #42181, #65434 ) ) ;
#29610=DIRECTION ( 'NONE',  ( 0.000000000000000000, 0.000000000000000000, 1.000000000000000000 ) ) ;
#29611=CARTESIAN_POINT ( 'NONE',  ( 0.1999999999999562961, 2.500000000000000000, 4.676537180435972552 ) ) ;
#29612=ORIENTED_EDGE ( 'NONE', *, *, #8514, .F. ) ;
#29613=ORIENTED_EDGE ( 'NONE', *, *, #110149, .T. ) ;
#29614=DIRECTION ( 'NONE',  ( 0.000000000000000000, 1.000000000000000000, 0.000000000000000000 ) ) ;
#29615=LINE ( 'NONE', #49284, #420 ) ;
#29616=VERTEX_POINT ( 'NONE', #104084 ) ;
#29617=ADVANCED_FACE ( 'NONE', ( #54334 ), #92983, .T. ) ;
#29618=DIRECTION ( 'NONE',  ( 0.000000000000000000, 0.000000000000000000, -1.000000000000000000 ) ) ;
#29620=DIRECTION ( 'NONE',  ( -4.274815082592931898E-19, -0.9999939076577903929, -0.003490651415223739937 ) ) ;
#29621=AXIS2_PLACEMENT_3D ( 'NONE', #59584, #9805, #89659 ) ;
#29622=CARTESIAN_POINT ( 'NONE',  ( 0.8499999999999557909, 2.500000000000000000, -7.188010851410854052 ) ) ;
#29623=DIRECTION ( 'NONE',  ( 0.000000000000000000, -0.000000000000000000, 1.000000000000000000 ) ) ;
#29624=AXIS2_PLACEMENT_3D ( 'NONE', #54815, #77674, #125494 ) ;
#29625=EDGE_CURVE ( 'NONE', #41344, #67957, #3303, .T. ) ;
#29626=CONICAL_SURFACE ( 'NONE', #127825, 0.1000000000000002554, 0.003490658503988666988 ) ;
#29627=DIRECTION ( 'NONE',  ( -0.000000000000000000, 1.000000000000000000, -0.000000000000000000 ) ) ;
#29628=CARTESIAN_POINT ( 'NONE',  ( 5.449999999999936229, 2.500000000000000000, 6.495190528383297135 ) ) ;
#29629=EDGE_CURVE ( 'NONE', #127552, #54932, #99069, .T. ) ;
#29630=EDGE_CURVE ( 'NONE', #76614, #45205, #17468, .T. ) ;
#29631=CIRCLE ( 'NONE', #52613, 0.06509327318403741736 ) ;
#29632=ORIENTED_EDGE ( 'NONE', *, *, #75925, .T. ) ;
#29633=AXIS2_PLACEMENT_3D ( 'NONE', #93268, #6611, #66206 ) ;
#29634=EDGE_LOOP ( 'NONE', ( #40156, #80487 ) ) ;
#29635=EDGE_CURVE ( 'NONE', #44929, #61864, #76079, .T. ) ;
#29636=ORIENTED_EDGE ( 'NONE', *, *, #56586, .T. ) ;
#29637=ORIENTED_EDGE ( 'NONE', *, *, #59327, .T. ) ;
#29638=DIRECTION ( 'NONE',  ( 0.000000000000000000, 1.000000000000000000, 0.000000000000000000 ) ) ;
#29639=DIRECTION ( 'NONE',  ( 0.000000000000000000, 0.000000000000000000, 1.000000000000000000 ) ) ;
#29640=AXIS2_PLACEMENT_3D ( 'NONE', #104501, #107070, #78291 ) ;
#29641=CARTESIAN_POINT ( 'NONE',  ( -5.650000000000019895, 2.500000000000000000, 2.511473670974873507 ) ) ;
#29642=CIRCLE ( 'NONE', #125764, 0.1000000000000000472 ) ;
#29643=ORIENTED_EDGE ( 'NONE', *, *, #6028, .F. ) ;
#29644=FACE_BOUND ( 'NONE', #129282, .T. ) ;
#29645=VERTEX_POINT ( 'NONE', #73319 ) ;
#29646=CARTESIAN_POINT ( 'NONE',  ( 6.849999999999927702, 12.50000000000000000, 1.753560074763284016 ) ) ;
#29647=CARTESIAN_POINT ( 'NONE',  ( -9.350000000000006750, 2.500000000000000000, 1.818653347947321475 ) ) ;
#29648=EDGE_CURVE ( 'NONE', #53411, #63511, #42647, .T. ) ;
#29649=AXIS2_PLACEMENT_3D ( 'NONE', #25260, #34476, #74384 ) ;
#29650=EDGE_CURVE ( 'NONE', #117332, #51834, #59375, .T. ) ;
#29651=CARTESIAN_POINT ( 'NONE',  ( 8.949999999999921130, 2.500000000000000000, 1.918653347947321564 ) ) ;
#29652=ADVANCED_FACE ( 'NONE', ( #64789 ), #4949, .T. ) ;
#29653=DIRECTION ( 'NONE',  ( 0.000000000000000000, 1.000000000000000000, 0.000000000000000000 ) ) ;
#29654=DIRECTION ( 'NONE',  ( 0.000000000000000000, 0.000000000000000000, -1.000000000000000000 ) ) ;
#29655=DIRECTION ( 'NONE',  ( 0.000000000000000000, 0.000000000000000000, 1.000000000000000000 ) ) ;
#29656=FACE_OUTER_BOUND ( 'NONE', #100523, .T. ) ;
#29657=CARTESIAN_POINT ( 'NONE',  ( 8.149999999999920419, 2.500000000000000000, 6.148780366869520897 ) ) ;
#29658=CARTESIAN_POINT ( 'NONE',  ( -12.89999999999999147, 2.500000000000000000, 3.537306695894645081 ) ) ;
#29659=CARTESIAN_POINT ( 'NONE',  ( 7.899999999999924860, 12.50000000000000000, -4.265033745738164406 ) ) ;
#29660=ORIENTED_EDGE ( 'NONE', *, *, #46707, .F. ) ;
#29662=ORIENTED_EDGE ( 'NONE', *, *, #52156, .T. ) ;
#29663=ORIENTED_EDGE ( 'NONE', *, *, #25565, .T. ) ;
#29664=FACE_OUTER_BOUND ( 'NONE', #49914, .T. ) ;
#29665=DIRECTION ( 'NONE',  ( 0.000000000000000000, 0.000000000000000000, 1.000000000000000000 ) ) ;
#29666=ORIENTED_EDGE ( 'NONE', *, *, #74680, .T. ) ;
#29667=ORIENTED_EDGE ( 'NONE', *, *, #98583, .T. ) ;
#29668=VERTEX_POINT ( 'NONE', #125637 ) ;
#29669=DIRECTION ( 'NONE',  ( -0.000000000000000000, 1.000000000000000000, -0.000000000000000000 ) ) ;
#29670=AXIS2_PLACEMENT_3D ( 'NONE', #102497, #52115, #2336 ) ;
#29671=CIRCLE ( 'NONE', #52641, 0.06509327318403745899 ) ;
#29672=PLANE ( 'NONE',  #101106 ) ;
#29673=FACE_OUTER_BOUND ( 'NONE', #77778, .T. ) ;
#29674=DIRECTION ( 'NONE',  ( 0.000000000000000000, 0.000000000000000000, 1.000000000000000000 ) ) ;
#29675=DIRECTION ( 'NONE',  ( 0.000000000000000000, -0.000000000000000000, 1.000000000000000000 ) ) ;
#29676=CARTESIAN_POINT ( 'NONE',  ( -4.250072516143177381E-14, 2.500000000000000000, -3.537306695894649966 ) ) ;
#29677=DIRECTION ( 'NONE',  ( 0.000000000000000000, -0.000000000000000000, 1.000000000000000000 ) ) ;
#29678=ORIENTED_EDGE ( 'NONE', *, *, #107155, .F. ) ;
#29679=CIRCLE ( 'NONE', #123739, 0.1000000000000002554 ) ;
#29680=AXIS2_PLACEMENT_3D ( 'NONE', #27742, #38232, #87306 ) ;
#29681=DIRECTION ( 'NONE',  ( 0.000000000000000000, -0.000000000000000000, 1.000000000000000000 ) ) ;
#29682=ORIENTED_EDGE ( 'NONE', *, *, #59128, .T. ) ;
#29683=CONICAL_SURFACE ( 'NONE', #59017, 0.1000000000000000056, 0.003490658503988666988 ) ;
#29684=ORIENTED_EDGE ( 'NONE', *, *, #106153, .T. ) ;
#29685=AXIS2_PLACEMENT_3D ( 'NONE', #73657, #114874, #3641 ) ;
#29686=EDGE_CURVE ( 'NONE', #7993, #1900, #5860, .T. ) ;
#29687=ORIENTED_EDGE ( 'NONE', *, *, #11465, .T. ) ;
#29688=CARTESIAN_POINT ( 'NONE',  ( -11.44999999999999751, 2.500000000000000000, -6.941600689897074794 ) ) ;
#29689=ORIENTED_EDGE ( 'NONE', *, *, #78158, .T. ) ;
#29690=EDGE_LOOP ( 'NONE', ( #128935, #86489, #45861, #32585 ) ) ;
#29691=AXIS2_PLACEMENT_3D ( 'NONE', #117311, #67591, #16550 ) ;
#29692=EDGE_CURVE ( 'NONE', #57270, #80732, #47110, .T. ) ;
#29693=DIRECTION ( 'NONE',  ( 0.000000000000000000, 0.000000000000000000, -1.000000000000000000 ) ) ;
#29694=CARTESIAN_POINT ( 'NONE',  ( -9.350000000000006750, 12.50000000000000000, -1.818653347947325916 ) ) ;
#29695=DIRECTION ( 'NONE',  ( 0.000000000000000000, -0.9999939076577903929, 0.003490651415223739937 ) ) ;
#29696=AXIS2_PLACEMENT_3D ( 'NONE', #108169, #9981, #70194 ) ;
#29697=CIRCLE ( 'NONE', #10878, 0.1000000000000000472 ) ;
#29698=DIRECTION ( 'NONE',  ( -0.000000000000000000, 1.000000000000000000, -0.000000000000000000 ) ) ;
#29699=CIRCLE ( 'NONE', #2572, 0.09999999999999982514 ) ;
#29700=ORIENTED_EDGE ( 'NONE', *, *, #70432, .F. ) ;
#29701=LINE ( 'NONE', #128576, #42826 ) ;
#29702=ORIENTED_EDGE ( 'NONE', *, *, #105961, .F. ) ;
#29703=FACE_OUTER_BOUND ( 'NONE', #76273, .T. ) ;
#29704=EDGE_LOOP ( 'NONE', ( #122495, #13515, #119140, #33190 ) ) ;
#29705=DIRECTION ( 'NONE',  ( -0.000000000000000000, 1.000000000000000000, -0.000000000000000000 ) ) ;
#29706=LINE ( 'NONE', #40180, #44110 ) ;
#29707=ORIENTED_EDGE ( 'NONE', *, *, #127512, .F. ) ;
#29708=CARTESIAN_POINT ( 'NONE',  ( -3.750000000000027534, 12.50000000000000000, -1.472243186433550122 ) ) ;
#29709=PLANE ( 'NONE',  #52017 ) ;
#29710=VERTEX_POINT ( 'NONE', #7149 ) ;
#29711=DIRECTION ( 'NONE',  ( 0.000000000000000000, 0.000000000000000000, -1.000000000000000000 ) ) ;
#29712=ORIENTED_EDGE ( 'NONE', *, *, #110607, .F. ) ;
#29713=VERTEX_POINT ( 'NONE', #126949 ) ;
#29714=FACE_OUTER_BOUND ( 'NONE', #6044, .T. ) ;
#29715=CARTESIAN_POINT ( 'NONE',  ( 6.649999999999930189, 2.500000000000000000, -2.857883832488653741 ) ) ;
#29717=CARTESIAN_POINT ( 'NONE',  ( 10.39999999999991154, 2.500000000000000000, 5.022947341949748790 ) ) ;
#29718=DIRECTION ( 'NONE',  ( 0.000000000000000000, 1.000000000000000000, 0.000000000000000000 ) ) ;
#29719=VERTEX_POINT ( 'NONE', #45814 ) ;
#29720=LINE ( 'NONE', #38266, #88485 ) ;
#29721=CONICAL_SURFACE ( 'NONE', #71577, 0.09999999999999982514, 0.003490658503988666988 ) ;
#29722=AXIS2_PLACEMENT_3D ( 'NONE', #121138, #1998, #92315 ) ;
#29723=ORIENTED_EDGE ( 'NONE', *, *, #6392, .F. ) ;
#29724=DIRECTION ( 'NONE',  ( 0.000000000000000000, -0.000000000000000000, 1.000000000000000000 ) ) ;
#29725=DIRECTION ( 'NONE',  ( 0.000000000000000000, 0.000000000000000000, -1.000000000000000000 ) ) ;
#29726=EDGE_CURVE ( 'NONE', #52060, #2207, #48382, .T. ) ;
#29727=CONICAL_SURFACE ( 'NONE', #79902, 0.09999999999999982514, 0.003490658503988666988 ) ;
#29729=AXIS2_PLACEMENT_3D ( 'NONE', #112596, #123056, #22296 ) ;
#29730=VECTOR ( 'NONE', #66359, 1000.000000000000000 ) ;
#29732=EDGE_CURVE ( 'NONE', #63696, #109777, #78144, .T. ) ;
#29733=CARTESIAN_POINT ( 'NONE',  ( -4.600000000000025402, 2.500000000000000000, -0.1000000000000023925 ) ) ;
#29734=CARTESIAN_POINT ( 'NONE',  ( -12.89999999999999325, 12.50000000000000000, -3.637306695894647390 ) ) ;
#29735=DIRECTION ( 'NONE',  ( 0.000000000000000000, 0.000000000000000000, 1.000000000000000000 ) ) ;
#29737=EDGE_CURVE ( 'NONE', #68264, #57867, #21701, .T. ) ;
#29738=CARTESIAN_POINT ( 'NONE',  ( 15.39999999999989200, 2.500000000000000000, 0.6928203230275494784 ) ) ;
#29739=VERTEX_POINT ( 'NONE', #106017 ) ;
#29740=AXIS2_PLACEMENT_3D ( 'NONE', #115012, #6332, #126136 ) ;
#29741=DIRECTION ( 'NONE',  ( 0.000000000000000000, 1.000000000000000000, 0.000000000000000000 ) ) ;
#29743=CARTESIAN_POINT ( 'NONE',  ( -4.800000000000022915, 12.50000000000000000, -0.3464101615137783474 ) ) ;
#29744=ADVANCED_FACE ( 'NONE', ( #116463 ), #44784, .T. ) ;
#29745=EDGE_CURVE ( 'NONE', #14967, #81450, #111577, .T. ) ;
#29746=EDGE_CURVE ( 'NONE', #27555, #72458, #85716, .T. ) ;
#29747=ORIENTED_EDGE ( 'NONE', *, *, #71294, .F. ) ;
#29748=DIRECTION ( 'NONE',  ( 0.000000000000000000, 0.000000000000000000, 1.000000000000000000 ) ) ;
#29749=ORIENTED_EDGE ( 'NONE', *, *, #6487, .F. ) ;
#29750=ORIENTED_EDGE ( 'NONE', *, *, #107036, .T. ) ;
#29751=DIRECTION ( 'NONE',  ( -4.274815082592931898E-19, -0.9999939076577903929, -0.003490651415223739937 ) ) ;
#29752=VERTEX_POINT ( 'NONE', #18906 ) ;
#29753=FACE_OUTER_BOUND ( 'NONE', #82929, .T. ) ;
#29754=DIRECTION ( 'NONE',  ( 0.000000000000000000, 0.000000000000000000, 1.000000000000000000 ) ) ;
#29755=CIRCLE ( 'NONE', #115504, 0.06509327318403745899 ) ;
#29756=ORIENTED_EDGE ( 'NONE', *, *, #99182, .T. ) ;
#29757=DIRECTION ( 'NONE',  ( -4.274815082592931898E-19, -0.9999939076577903929, -0.003490651415223739937 ) ) ;
#29758=DIRECTION ( 'NONE',  ( -4.274815082592931898E-19, -0.9999939076577903929, -0.003490651415223739937 ) ) ;
#29759=ORIENTED_EDGE ( 'NONE', *, *, #15762, .F. ) ;
#29760=CARTESIAN_POINT ( 'NONE',  ( -6.850000000000013856, 12.50000000000000000, 1.753560074763284016 ) ) ;
#29761=VECTOR ( 'NONE', #26545, 1000.000000000000000 ) ;
#29762=ORIENTED_EDGE ( 'NONE', *, *, #29246, .T. ) ;
#29763=CIRCLE ( 'NONE', #25540, 0.06509327318403745899 ) ;
#29764=AXIS2_PLACEMENT_3D ( 'NONE', #50570, #81339, #121255 ) ;
#29765=CIRCLE ( 'NONE', #36033, 0.06509327318403745899 ) ;
#29766=VERTEX_POINT ( 'NONE', #108590 ) ;
#29767=EDGE_LOOP ( 'NONE', ( #111938, #82639, #83200, #109096 ) ) ;
#29768=DIRECTION ( 'NONE',  ( -0.000000000000000000, -1.000000000000000000, -0.000000000000000000 ) ) ;
#29770=DIRECTION ( 'NONE',  ( 0.000000000000000000, 0.000000000000000000, -1.000000000000000000 ) ) ;
#29771=FACE_BOUND ( 'NONE', #17621, .T. ) ;
#29772=ORIENTED_EDGE ( 'NONE', *, *, #50141, .T. ) ;
#29773=CARTESIAN_POINT ( 'NONE',  ( 12.29999999999990301, 12.50000000000000000, -0.3464101615137782364 ) ) ;
#29774=CARTESIAN_POINT ( 'NONE',  ( 3.549999999999943867, 2.500000000000000000, -6.248780366869526759 ) ) ;
#29775=CIRCLE ( 'NONE', #4606, 0.1000000000000002554 ) ;
#29776=ORIENTED_EDGE ( 'NONE', *, *, #94585, .T. ) ;
#29777=AXIS2_PLACEMENT_3D ( 'NONE', #80660, #49275, #121859 ) ;
#29778=CARTESIAN_POINT ( 'NONE',  ( -0.4500000000000397571, 12.50000000000000000, -6.495190528383302464 ) ) ;
#29779=LINE ( 'NONE', #127979, #3156 ) ;
#29780=AXIS2_PLACEMENT_3D ( 'NONE', #113223, #3284, #12444 ) ;
#29781=CONICAL_SURFACE ( 'NONE', #40255, 0.1000000000000002554, 0.003490658503988666988 ) ;
#29782=AXIS2_PLACEMENT_3D ( 'NONE', #94363, #125128, #15800 ) ;
#29783=CARTESIAN_POINT ( 'NONE',  ( -5.000000000000023093, 12.50000000000000000, 5.022947341949748790 ) ) ;
#29784=EDGE_CURVE ( 'NONE', #35476, #117024, #127589, .T. ) ;
#29785=DIRECTION ( 'NONE',  ( 0.000000000000000000, 1.000000000000000000, 0.000000000000000000 ) ) ;
#29786=DIRECTION ( 'NONE',  ( 0.000000000000000000, 0.000000000000000000, -1.000000000000000000 ) ) ;
#29787=EDGE_CURVE ( 'NONE', #78590, #12380, #82447, .T. ) ;
#29788=CARTESIAN_POINT ( 'NONE',  ( -2.100000000000033396, 12.50000000000000000, -0.6928203230275542523 ) ) ;
#29789=CARTESIAN_POINT ( 'NONE',  ( -14.34999999999998543, 12.50000000000000000, -2.511473670974875727 ) ) ;
#29790=EDGE_CURVE ( 'NONE', #60953, #22036, #18271, .T. ) ;
#29791=VERTEX_POINT ( 'NONE', #38588 ) ;
#29792=VECTOR ( 'NONE', #111908, 1000.000000000000000 ) ;
#29793=ORIENTED_EDGE ( 'NONE', *, *, #32603, .T. ) ;
#29794=ORIENTED_EDGE ( 'NONE', *, *, #37934, .F. ) ;
#29795=EDGE_LOOP ( 'NONE', ( #110166, #31548 ) ) ;
#29796=ORIENTED_EDGE ( 'NONE', *, *, #84103, .F. ) ;
#29797=PLANE ( 'NONE',  #104847 ) ;
#29798=EDGE_CURVE ( 'NONE', #99999, #80146, #61514, .T. ) ;
#29799=DIRECTION ( 'NONE',  ( -4.274815082592931898E-19, -0.9999939076577903929, -0.003490651415223739937 ) ) ;
#29800=ORIENTED_EDGE ( 'NONE', *, *, #127484, .T. ) ;
#29801=ADVANCED_FACE ( 'NONE', ( #26169 ), #95553, .T. ) ;
#29802=FACE_BOUND ( 'NONE', #94651, .T. ) ;
#29803=CARTESIAN_POINT ( 'NONE',  ( 8.149999999999923972, 2.500000000000000000, 1.918653347947321564 ) ) ;
#29804=ADVANCED_FACE ( 'NONE', ( #47747 ), #17563, .T. ) ;
#29805=EDGE_CURVE ( 'NONE', #89331, #42654, #56261, .T. ) ;
#29806=EDGE_CURVE ( 'NONE', #7162, #107859, #28753, .T. ) ;
#29808=DIRECTION ( 'NONE',  ( 0.000000000000000000, 0.000000000000000000, 1.000000000000000000 ) ) ;
#29809=LINE ( 'NONE', #81489, #37036 ) ;
#29810=CARTESIAN_POINT ( 'NONE',  ( 2.099999999999950351, 12.50000000000000000, -2.276824562219559311E-15 ) ) ;
#29811=AXIS2_PLACEMENT_3D ( 'NONE', #89763, #121790, #72076 ) ;
#29812=DIRECTION ( 'NONE',  ( -0.000000000000000000, 1.000000000000000000, -0.000000000000000000 ) ) ;
#29813=ORIENTED_EDGE ( 'NONE', *, *, #32810, .T. ) ;
#29814=EDGE_CURVE ( 'NONE', #34970, #39517, #126340, .T. ) ;
#29815=ORIENTED_EDGE ( 'NONE', *, *, #85425, .T. ) ;
#29816=ORIENTED_EDGE ( 'NONE', *, *, #63486, .F. ) ;
#29817=VERTEX_POINT ( 'NONE', #36651 ) ;
#29818=ORIENTED_EDGE ( 'NONE', *, *, #10867, .F. ) ;
#29819=AXIS2_PLACEMENT_3D ( 'NONE', #124971, #5815, #76518 ) ;
#29820=CARTESIAN_POINT ( 'NONE',  ( 13.39053294304986785, 2.500000000000000888, 7.037281287790724704 ) ) ;
#29821=DIRECTION ( 'NONE',  ( -0.000000000000000000, 1.000000000000000000, -0.000000000000000000 ) ) ;
#29822=EDGE_LOOP ( 'NONE', ( #70313, #56686 ) ) ;
#29823=DIRECTION ( 'NONE',  ( 0.000000000000000000, 0.000000000000000000, 1.000000000000000000 ) ) ;
#29824=DIRECTION ( 'NONE',  ( 0.000000000000000000, 0.000000000000000000, 1.000000000000000000 ) ) ;
#29825=CONICAL_SURFACE ( 'NONE', #61122, 0.1000000000000000472, 0.003490658503988666988 ) ;
#29826=VECTOR ( 'NONE', #11034, 1000.000000000000000 ) ;
#29827=CIRCLE ( 'NONE', #113443, 0.09999999999999982514 ) ;
#29828=FACE_OUTER_BOUND ( 'NONE', #108215, .T. ) ;
#29830=FACE_OUTER_BOUND ( 'NONE', #43733, .T. ) ;
#29831=PLANE ( 'NONE',  #86468 ) ;
#29832=AXIS2_PLACEMENT_3D ( 'NONE', #96778, #16907, #42740 ) ;
#29833=AXIS2_PLACEMENT_3D ( 'NONE', #41785, #122265, #101974 ) ;
#29834=DIRECTION ( 'NONE',  ( 0.000000000000000000, 1.000000000000000000, 0.000000000000000000 ) ) ;
#29835=ORIENTED_EDGE ( 'NONE', *, *, #118396, .T. ) ;
#29836=DIRECTION ( 'NONE',  ( 0.000000000000000000, 1.000000000000000000, 0.000000000000000000 ) ) ;
#29837=AXIS2_PLACEMENT_3D ( 'NONE', #79618, #87486, #98590 ) ;
#29838=EDGE_LOOP ( 'NONE', ( #91463, #23219, #96410, #12105 ) ) ;
#29839=ORIENTED_EDGE ( 'NONE', *, *, #11476, .F. ) ;
#29840=DIRECTION ( 'NONE',  ( -4.274815082592931898E-19, -0.9999939076577903929, -0.003490651415223739937 ) ) ;
#29841=DIRECTION ( 'NONE',  ( 0.000000000000000000, 1.000000000000000000, 0.000000000000000000 ) ) ;
#29842=DIRECTION ( 'NONE',  ( 0.000000000000000000, 1.000000000000000000, 0.000000000000000000 ) ) ;
#29843=ORIENTED_EDGE ( 'NONE', *, *, #57091, .F. ) ;
#29844=ORIENTED_EDGE ( 'NONE', *, *, #109467, .T. ) ;
#29845=CIRCLE ( 'NONE', #46551, 0.09999999999999982514 ) ;
#29846=CARTESIAN_POINT ( 'NONE',  ( 1.049999999999954525, 2.500000000000000000, 1.718653347947321386 ) ) ;
#29847=EDGE_CURVE ( 'NONE', #76431, #64157, #128904, .T. ) ;
#29848=CARTESIAN_POINT ( 'NONE',  ( -2.100000000000033840, 12.50000000000000000, 5.022947341949748790 ) ) ;
#29849=DIRECTION ( 'NONE',  ( 0.000000000000000000, 0.000000000000000000, -1.000000000000000000 ) ) ;
#29850=DIRECTION ( 'NONE',  ( 0.000000000000000000, 1.000000000000000000, 0.000000000000000000 ) ) ;
#29851=VERTEX_POINT ( 'NONE', #119687 ) ;
#29852=CARTESIAN_POINT ( 'NONE',  ( -10.65000000000000391, 12.50000000000000000, -2.446380397790836270 ) ) ;
#29853=CONICAL_SURFACE ( 'NONE', #109259, 0.1000000000000002554, 0.003490658503988666988 ) ;
#29855=DIRECTION ( 'NONE',  ( 0.000000000000000000, 1.000000000000000000, 0.000000000000000000 ) ) ;
#29856=AXIS2_PLACEMENT_3D ( 'NONE', #53780, #83258, #110761 ) ;
#29857=VERTEX_POINT ( 'NONE', #120355 ) ;
#29858=LINE ( 'NONE', #109715, #100573 ) ;
#29859=DIRECTION ( 'NONE',  ( 0.000000000000000000, -0.000000000000000000, 1.000000000000000000 ) ) ;
#29861=FACE_OUTER_BOUND ( 'NONE', #94594, .T. ) ;
#29862=CIRCLE ( 'NONE', #25734, 0.1000000000000002554 ) ;
#29863=ORIENTED_EDGE ( 'NONE', *, *, #95191, .T. ) ;
#29864=AXIS2_PLACEMENT_3D ( 'NONE', #25659, #34217, #13900 ) ;
#29865=CIRCLE ( 'NONE', #11060, 0.09999999999999982514 ) ;
#29866=CARTESIAN_POINT ( 'NONE',  ( -1.050000000000038680, 2.500000000000000000, 2.511473670974873507 ) ) ;
#29867=CIRCLE ( 'NONE', #6846, 0.06509327318403745899 ) ;
#29868=ORIENTED_EDGE ( 'NONE', *, *, #51221, .F. ) ;
#29869=VERTEX_POINT ( 'NONE', #98756 ) ;
#29870=CARTESIAN_POINT ( 'NONE',  ( 8.349999999999923261, 2.500000000000000000, -7.188010851410854052 ) ) ;
#29871=DIRECTION ( 'NONE',  ( -0.000000000000000000, -1.000000000000000000, -0.000000000000000000 ) ) ;
#29872=PLANE ( 'NONE',  #78344 ) ;
#29874=CIRCLE ( 'NONE', #19391, 0.1000000000000002554 ) ;
#29875=DIRECTION ( 'NONE',  ( 0.000000000000000000, 0.000000000000000000, 1.000000000000000000 ) ) ;
#29876=CARTESIAN_POINT ( 'NONE',  ( -1.650000000000035216, 2.500000000000000000, -5.802370205355749988 ) ) ;
#29877=AXIS2_PLACEMENT_3D ( 'NONE', #102230, #32861, #82595 ) ;
#29878=DIRECTION ( 'NONE',  ( -0.000000000000000000, -1.000000000000000000, -0.000000000000000000 ) ) ;
#29879=CIRCLE ( 'NONE', #71832, 0.09999999999999982514 ) ;
#29880=CARTESIAN_POINT ( 'NONE',  ( -11.84999999999999787, 12.50000000000000000, -6.083687093685485436 ) ) ;
#29881=CONICAL_SURFACE ( 'NONE', #103023, 0.09999999999999982514, 0.003490658503988666988 ) ;
#29882=PLANE ( 'NONE',  #63077 ) ;
#29883=CIRCLE ( 'NONE', #86292, 0.06509327318403745899 ) ;
#29884=EDGE_CURVE ( 'NONE', #54255, #117981, #58848, .T. ) ;
#29885=AXIS2_PLACEMENT_3D ( 'NONE', #50908, #52187, #20796 ) ;
#29886=ORIENTED_EDGE ( 'NONE', *, *, #49034, .T. ) ;
#29887=FACE_OUTER_BOUND ( 'NONE', #2144, .T. ) ;
#29888=DIRECTION ( 'NONE',  ( 0.000000000000000000, 0.000000000000000000, 1.000000000000000000 ) ) ;
#29889=CARTESIAN_POINT ( 'NONE',  ( 1.249999999999954259, 2.500000000000000000, -7.188010851410854052 ) ) ;
#29891=CARTESIAN_POINT ( 'NONE',  ( -6.900000000000019007, 12.50000000000000000, 0.3464101615137735735 ) ) ;
#29892=EDGE_CURVE ( 'NONE', #108388, #8747, #60784, .T. ) ;
#29893=VERTEX_POINT ( 'NONE', #30697 ) ;
#29894=CARTESIAN_POINT ( 'NONE',  ( 13.94999999999989626, 12.50000000000000000, 2.511473670974873507 ) ) ;
#29895=FACE_OUTER_BOUND ( 'NONE', #43198, .T. ) ;
#29896=DIRECTION ( 'NONE',  ( 0.000000000000000000, 1.000000000000000000, 0.000000000000000000 ) ) ;
#29897=ORIENTED_EDGE ( 'NONE', *, *, #60469, .F. ) ;
#29898=EDGE_CURVE ( 'NONE', #116919, #100324, #117921, .T. ) ;
#29899=EDGE_CURVE ( 'NONE', #122002, #80402, #9269, .T. ) ;
#29900=AXIS2_PLACEMENT_3D ( 'NONE', #109367, #19708, #121122 ) ;
#29901=CIRCLE ( 'NONE', #36174, 0.06509327318403745899 ) ;
#29902=ADVANCED_FACE ( 'NONE', ( #88956 ), #59523, .T. ) ;
#29903=ADVANCED_FACE ( 'NONE', ( #91532 ), #5048, .T. ) ;
#29904=EDGE_CURVE ( 'NONE', #18510, #47774, #49049, .T. ) ;
#29905=ORIENTED_EDGE ( 'NONE', *, *, #1340, .T. ) ;
#29906=LINE ( 'NONE', #109756, #787 ) ;
#29907=CIRCLE ( 'NONE', #55235, 0.1000000000000002554 ) ;
#29908=VERTEX_POINT ( 'NONE', #119060 ) ;
#29909=EDGE_LOOP ( 'NONE', ( #68621, #95232, #118014, #44781 ) ) ;
#29910=ORIENTED_EDGE ( 'NONE', *, *, #127498, .F. ) ;
#29911=DIRECTION ( 'NONE',  ( 0.000000000000000000, 0.000000000000000000, 1.000000000000000000 ) ) ;
#29912=AXIS2_PLACEMENT_3D ( 'NONE', #12267, #73138, #90840 ) ;
#29913=AXIS2_PLACEMENT_3D ( 'NONE', #120824, #83493, #122759 ) ;
#29914=ADVANCED_FACE ( 'NONE', ( #51617 ), #128424, .T. ) ;
#29915=DIRECTION ( 'NONE',  ( 0.000000000000000000, 0.000000000000000000, 1.000000000000000000 ) ) ;
#29916=CARTESIAN_POINT ( 'NONE',  ( 9.799999999999913669, 2.500000000000000000, -3.883716857408426648 ) ) ;
#29918=CIRCLE ( 'NONE', #96795, 0.1000000000000002554 ) ;
#29919=ADVANCED_FACE ( 'NONE', ( #111144 ), #89599, .T. ) ;
#29920=VERTEX_POINT ( 'NONE', #109218 ) ;
#29921=AXIS2_PLACEMENT_3D ( 'NONE', #37148, #27298, #17473 ) ;
#29922=CONICAL_SURFACE ( 'NONE', #71777, 0.09999999999999982514, 0.003490658503988666988 ) ;
#29923=CARTESIAN_POINT ( 'NONE',  ( 2.099999999999948574, 2.500000000000000000, 3.637306695894644726 ) ) ;
#29924=AXIS2_PLACEMENT_3D ( 'NONE', #28711, #77783, #68616 ) ;
#29925=ORIENTED_EDGE ( 'NONE', *, *, #91255, .F. ) ;
#29926=CARTESIAN_POINT ( 'NONE',  ( 11.24999999999994316, 12.50000000000000000, 2.099970236277060032 ) ) ;
#29928=FACE_OUTER_BOUND ( 'NONE', #56510, .T. ) ;
#29929=LINE ( 'NONE', #117625, #124940 ) ;
#29932=ORIENTED_EDGE ( 'NONE', *, *, #7719, .T. ) ;
#29933=VERTEX_POINT ( 'NONE', #19566 ) ;
#29934=VERTEX_POINT ( 'NONE', #50978 ) ;
#29936=FACE_OUTER_BOUND ( 'NONE', #119854, .T. ) ;
#29937=DIRECTION ( 'NONE',  ( 0.000000000000000000, -0.9999939076577903929, 0.003490651415223739937 ) ) ;
#29938=DIRECTION ( 'NONE',  ( 0.000000000000000000, 0.000000000000000000, 1.000000000000000000 ) ) ;
#29939=FACE_BOUND ( 'NONE', #12342, .T. ) ;
#29940=DIRECTION ( 'NONE',  ( 0.000000000000000000, -0.9999939076577903929, 0.003490651415223739937 ) ) ;
#29942=DIRECTION ( 'NONE',  ( -0.000000000000000000, -1.000000000000000000, -0.000000000000000000 ) ) ;
#29943=DIRECTION ( 'NONE',  ( -0.000000000000000000, -1.000000000000000000, -0.000000000000000000 ) ) ;
#29944=AXIS2_PLACEMENT_3D ( 'NONE', #30907, #70808, #30267 ) ;
#29945=DIRECTION ( 'NONE',  ( 0.000000000000000000, -0.9999939076577903929, 0.003490651415223739937 ) ) ;
#29946=DIRECTION ( 'NONE',  ( 0.000000000000000000, 0.000000000000000000, 1.000000000000000000 ) ) ;
#29947=EDGE_CURVE ( 'NONE', #42572, #73565, #13455, .T. ) ;
#29948=CARTESIAN_POINT ( 'NONE',  ( 3.949999999999938893, 12.50000000000000000, 6.148780366869520009 ) ) ;
#29949=CIRCLE ( 'NONE', #53026, 0.06509327318403745899 ) ;
#29950=ADVANCED_FACE ( 'NONE', ( #90883 ), #111676, .T. ) ;
#29951=AXIS2_PLACEMENT_3D ( 'NONE', #110906, #43486, #90634 ) ;
#29952=CIRCLE ( 'NONE', #61255, 0.06509327318403745899 ) ;
#29953=DIRECTION ( 'NONE',  ( 0.000000000000000000, 0.000000000000000000, -1.000000000000000000 ) ) ;
#29954=EDGE_CURVE ( 'NONE', #98108, #56262, #23853, .T. ) ;
#29955=ORIENTED_EDGE ( 'NONE', *, *, #43095, .F. ) ;
#29956=EDGE_LOOP ( 'NONE', ( #11064, #52242, #97116, #56553 ) ) ;
#29957=VERTEX_POINT ( 'NONE', #11674 ) ;
#29958=ORIENTED_EDGE ( 'NONE', *, *, #114050, .T. ) ;
#29959=CARTESIAN_POINT ( 'NONE',  ( -12.89999999999999147, 2.500000000000000000, 3.637306695894644726 ) ) ;
#29960=FACE_OUTER_BOUND ( 'NONE', #99903, .T. ) ;
#29961=ADVANCED_FACE ( 'NONE', ( #30044 ), #80380, .T. ) ;
#29962=FACE_BOUND ( 'NONE', #49907, .T. ) ;
#29963=AXIS2_PLACEMENT_3D ( 'NONE', #96096, #86259, #96727 ) ;
#29964=CIRCLE ( 'NONE', #103110, 0.09999999999999982514 ) ;
#29965=FACE_OUTER_BOUND ( 'NONE', #12159, .T. ) ;
#29966=ADVANCED_FACE ( 'NONE', ( #109886 ), #78234, .T. ) ;
#29967=AXIS2_PLACEMENT_3D ( 'NONE', #78943, #107080, #87443 ) ;
#29968=AXIS2_PLACEMENT_3D ( 'NONE', #43920, #22351, #22985 ) ;
#29969=ADVANCED_FACE ( 'NONE', ( #90219 ), #11325, .T. ) ;
#29970=VERTEX_POINT ( 'NONE', #22170 ) ;
#29971=CARTESIAN_POINT ( 'NONE',  ( 12.89999999999990088, 12.50000000000000000, -4.395220292106239768 ) ) ;
#29972=DIRECTION ( 'NONE',  ( -0.000000000000000000, -1.000000000000000000, -0.000000000000000000 ) ) ;
#29973=DIRECTION ( 'NONE',  ( 0.000000000000000000, 0.000000000000000000, 1.000000000000000000 ) ) ;
#29974=FACE_OUTER_BOUND ( 'NONE', #83763, .T. ) ;
#29975=ORIENTED_EDGE ( 'NONE', *, *, #92069, .T. ) ;
#29976=CARTESIAN_POINT ( 'NONE',  ( -12.04999999999999538, 2.500000000000000000, 6.395190528383296602 ) ) ;
#29977=ADVANCED_FACE ( 'NONE', ( #112471 ), #86619, .T. ) ;
#29978=AXIS2_PLACEMENT_3D ( 'NONE', #18640, #98479, #8808 ) ;
#29979=VECTOR ( 'NONE', #16000, 1000.000000000000000 ) ;
#29980=CIRCLE ( 'NONE', #57052, 0.06509327318403745899 ) ;
#29981=ORIENTED_EDGE ( 'NONE', *, *, #30997, .F. ) ;
#29982=EDGE_LOOP ( 'NONE', ( #109511, #47393, #36221, #41974 ) ) ;
#29983=DIRECTION ( 'NONE',  ( 0.000000000000000000, 0.000000000000000000, 1.000000000000000000 ) ) ;
#29984=CARTESIAN_POINT ( 'NONE',  ( 1.249999999999988454, 12.50000000000000000, -2.165063509461101710 ) ) ;
#29985=VECTOR ( 'NONE', #62497, 1000.000000000000000 ) ;
#29986=ORIENTED_EDGE ( 'NONE', *, *, #17170, .F. ) ;
#29987=DIRECTION ( 'NONE',  ( 0.000000000000000000, 0.000000000000000000, 1.000000000000000000 ) ) ;
#29988=LINE ( 'NONE', #15954, #104271 ) ;
#29989=ORIENTED_EDGE ( 'NONE', *, *, #16324, .T. ) ;
#29990=FACE_OUTER_BOUND ( 'NONE', #15126, .T. ) ;
#29991=EDGE_LOOP ( 'NONE', ( #43650, #49783, #64579, #30536 ) ) ;
#29992=FACE_OUTER_BOUND ( 'NONE', #85439, .T. ) ;
#29993=EDGE_CURVE ( 'NONE', #92156, #81635, #71976, .T. ) ;
#29994=ORIENTED_EDGE ( 'NONE', *, *, #14298, .F. ) ;
#29995=DIRECTION ( 'NONE',  ( -0.000000000000000000, -1.000000000000000000, -0.000000000000000000 ) ) ;
#29996=ORIENTED_EDGE ( 'NONE', *, *, #98032, .T. ) ;
#29998=VERTEX_POINT ( 'NONE', #44354 ) ;
#29999=DIRECTION ( 'NONE',  ( -0.000000000000000000, -1.000000000000000000, -0.000000000000000000 ) ) ;
#30000=CARTESIAN_POINT ( 'NONE',  ( 4.599999999999938360, 2.500000000000000000, -0.7928203230275542301 ) ) ;
#30001=AXIS2_PLACEMENT_3D ( 'NONE', #84418, #26790, #85059 ) ;
#30002=DIRECTION ( 'NONE',  ( -0.000000000000000000, -1.000000000000000000, -0.000000000000000000 ) ) ;
#30003=AXIS2_PLACEMENT_3D ( 'NONE', #119483, #108381, #78300 ) ;
#30004=CARTESIAN_POINT ( 'NONE',  ( 0.1999999999999562961, 2.500000000000000000, 4.576537180435972019 ) ) ;
#30005=CARTESIAN_POINT ( 'NONE',  ( -4.999999999999986677, 2.500000000000000000, 0.09999999999999772959 ) ) ;
#30006=ORIENTED_EDGE ( 'NONE', *, *, #73288, .F. ) ;
#30007=ORIENTED_EDGE ( 'NONE', *, *, #21073, .F. ) ;
#30008=VERTEX_POINT ( 'NONE', #22811 ) ;
#30009=PLANE ( 'NONE',  #129101 ) ;
#30010=VECTOR ( 'NONE', #67511, 1000.000000000000000 ) ;
#30011=EDGE_CURVE ( 'NONE', #90336, #78915, #43745, .T. ) ;
#30013=CONICAL_SURFACE ( 'NONE', #48894, 0.1000000000000002554, 0.003490658503988666988 ) ;
#30014=CONICAL_SURFACE ( 'NONE', #65490, 0.1000000000000002554, 0.003490658503988666988 ) ;
#30015=DIRECTION ( 'NONE',  ( 0.000000000000000000, -0.9999939076577903929, 0.003490651415223739937 ) ) ;
#30016=VERTEX_POINT ( 'NONE', #74470 ) ;
#30017=ORIENTED_EDGE ( 'NONE', *, *, #35361, .T. ) ;
#30018=ORIENTED_EDGE ( 'NONE', *, *, #32447, .F. ) ;
#30019=LINE ( 'NONE', #58194, #74911 ) ;
#30021=CARTESIAN_POINT ( 'NONE',  ( 12.89999999999990088, 2.500000000000000000, -4.330127018922201643 ) ) ;
#30022=AXIS2_PLACEMENT_3D ( 'NONE', #121274, #21803, #62996 ) ;
#30023=CIRCLE ( 'NONE', #27949, 0.09999999999999982514 ) ;
#30024=DIRECTION ( 'NONE',  ( -0.000000000000000000, 1.000000000000000000, -0.000000000000000000 ) ) ;
#30025=DIRECTION ( 'NONE',  ( 0.000000000000000000, 0.000000000000000000, -1.000000000000000000 ) ) ;
#30026=LINE ( 'NONE', #38569, #82102 ) ;
#30027=AXIS2_PLACEMENT_3D ( 'NONE', #37090, #49502, #109697 ) ;
#30028=DIRECTION ( 'NONE',  ( 0.000000000000000000, 0.000000000000000000, -1.000000000000000000 ) ) ;
#30029=DIRECTION ( 'NONE',  ( 0.000000000000000000, 1.000000000000000000, 0.000000000000000000 ) ) ;
#30030=VECTOR ( 'NONE', #49205, 1000.000000000000000 ) ;
#30031=ADVANCED_FACE ( 'NONE', ( #101999 ), #48993, .T. ) ;
#30032=CARTESIAN_POINT ( 'NONE',  ( -4.150000000000024336, 2.500000000000000000, -2.165063509461101710 ) ) ;
#30033=ORIENTED_EDGE ( 'NONE', *, *, #111064, .T. ) ;
#30034=VERTEX_POINT ( 'NONE', #92165 ) ;
#30035=FACE_OUTER_BOUND ( 'NONE', #27419, .T. ) ;
#30036=VERTEX_POINT ( 'NONE', #33898 ) ;
#30037=VERTEX_POINT ( 'NONE', #122293 ) ;
#30039=CARTESIAN_POINT ( 'NONE',  ( 12.49999999999990585, 2.500000000000000000, 3.737306695894644371 ) ) ;
#30040=PLANE ( 'NONE',  #100112 ) ;
#30041=AXIS2_PLACEMENT_3D ( 'NONE', #3993, #33483, #83842 ) ;
#30042=DIRECTION ( 'NONE',  ( -0.000000000000000000, 1.000000000000000000, -0.000000000000000000 ) ) ;
#30043=FACE_OUTER_BOUND ( 'NONE', #31071, .T. ) ;
#30044=FACE_OUTER_BOUND ( 'NONE', #57709, .T. ) ;
#30045=LINE ( 'NONE', #52900, #83271 ) ;
#30046=VECTOR ( 'NONE', #14115, 1000.000000000000000 ) ;
#30047=DIRECTION ( 'NONE',  ( -0.000000000000000000, -1.000000000000000000, -0.000000000000000000 ) ) ;
#30048=CIRCLE ( 'NONE', #48831, 0.06509327318403745899 ) ;
#30049=AXIS2_PLACEMENT_3D ( 'NONE', #5589, #124742, #56622 ) ;
#30050=ORIENTED_EDGE ( 'NONE', *, *, #75952, .T. ) ;
#30051=ADVANCED_FACE ( 'NONE', ( #64004 ), #63658, .T. ) ;
#30052=ORIENTED_EDGE ( 'NONE', *, *, #127897, .T. ) ;
#30053=VERTEX_POINT ( 'NONE', #123549 ) ;
#30054=ORIENTED_EDGE ( 'NONE', *, *, #9936, .T. ) ;
#30055=AXIS2_PLACEMENT_3D ( 'NONE', #114442, #117005, #94813 ) ;
#30056=DIRECTION ( 'NONE',  ( 0.000000000000000000, 0.000000000000000000, 1.000000000000000000 ) ) ;
#30057=DIRECTION ( 'NONE',  ( -0.000000000000000000, 1.000000000000000000, -0.000000000000000000 ) ) ;
#30058=VECTOR ( 'NONE', #71721, 1000.000000000000000 ) ;
#30059=CIRCLE ( 'NONE', #103204, 0.1000000000000002554 ) ;
#30060=EDGE_CURVE ( 'NONE', #100762, #3469, #65693, .T. ) ;
#30061=ORIENTED_EDGE ( 'NONE', *, *, #28602, .F. ) ;
#30062=DIRECTION ( 'NONE',  ( -0.000000000000000000, -1.000000000000000000, -0.000000000000000000 ) ) ;
#30063=CIRCLE ( 'NONE', #53128, 0.1000000000000000472 ) ;
#30064=CARTESIAN_POINT ( 'NONE',  ( -10.85000000000000142, 12.50000000000000000, -1.407149913249508666 ) ) ;
#30065=CARTESIAN_POINT ( 'NONE',  ( -4.600000000000024514, 2.500000000000000000, 5.122947341949749323 ) ) ;
#30066=CARTESIAN_POINT ( 'NONE',  ( 6.049999999999934097, 12.50000000000000000, 6.083687093685483660 ) ) ;
#30067=ORIENTED_EDGE ( 'NONE', *, *, #112844, .F. ) ;
#30068=ADVANCED_FACE ( 'NONE', ( #32643 ), #52254, .T. ) ;
#30070=EDGE_CURVE ( 'NONE', #60798, #17292, #124212, .T. ) ;
#30071=CARTESIAN_POINT ( 'NONE',  ( -9.600000000000006750, 2.500000000000000000, 5.022947341949748790 ) ) ;
#30072=CIRCLE ( 'NONE', #78186, 0.09999999999999982514 ) ;
#30073=EDGE_CURVE ( 'NONE', #7948, #24838, #115966, .T. ) ;
#30074=DIRECTION ( 'NONE',  ( 0.000000000000000000, 0.000000000000000000, 1.000000000000000000 ) ) ;
#30075=ORIENTED_EDGE ( 'NONE', *, *, #50637, .T. ) ;
#30076=CIRCLE ( 'NONE', #4998, 0.06509327318403745899 ) ;
#30077=EDGE_CURVE ( 'NONE', #74262, #79739, #53288, .T. ) ;
#30078=CONICAL_SURFACE ( 'NONE', #80244, 0.1000000000000002554, 0.003490658503988666988 ) ;
#30079=ORIENTED_EDGE ( 'NONE', *, *, #58416, .T. ) ;
#30080=ADVANCED_FACE ( 'NONE', ( #124859 ), #24035, .T. ) ;
#30081=ORIENTED_EDGE ( 'NONE', *, *, #26089, .T. ) ;
#30082=EDGE_LOOP ( 'NONE', ( #16188, #12434 ) ) ;
#30083=CARTESIAN_POINT ( 'NONE',  ( 10.79999999999991012, 2.500000000000000000, 4.330127018922196314 ) ) ;
#30084=AXIS2_PLACEMENT_3D ( 'NONE', #27691, #67614, #107561 ) ;
#30085=EDGE_CURVE ( 'NONE', #51302, #96401, #94106, .T. ) ;
#30086=FACE_OUTER_BOUND ( 'NONE', #128327, .T. ) ;
#30087=DIRECTION ( 'NONE',  ( 0.000000000000000000, 0.000000000000000000, 1.000000000000000000 ) ) ;
#30088=CONICAL_SURFACE ( 'NONE', #78095, 0.1000000000000000472, 0.003490658503988666988 ) ;
#30089=EDGE_CURVE ( 'NONE', #110807, #57482, #38623, .T. ) ;
#30090=EDGE_CURVE ( 'NONE', #83674, #35537, #80480, .T. ) ;
#30091=CARTESIAN_POINT ( 'NONE',  ( -9.800000000000006040, 12.50000000000000000, 4.676537180435972552 ) ) ;
#30092=ORIENTED_EDGE ( 'NONE', *, *, #46893, .F. ) ;
#30093=CARTESIAN_POINT ( 'NONE',  ( 11.44999999999990870, 12.50000000000000000, 6.776507416713035248 ) ) ;
#30094=CARTESIAN_POINT ( 'NONE',  ( 14.34999999999989306, 12.50000000000000000, -1.753560074763288679 ) ) ;
#30095=CARTESIAN_POINT ( 'NONE',  ( -8.300000000000009592, 2.500000000000000000, 4.330127018922196314 ) ) ;
#30096=DIRECTION ( 'NONE',  ( 0.000000000000000000, 0.000000000000000000, 1.000000000000000000 ) ) ;
#30097=ADVANCED_FACE ( 'NONE', ( #12947 ), #52899, .T. ) ;
#30098=ORIENTED_EDGE ( 'NONE', *, *, #126529, .T. ) ;
#30099=FACE_OUTER_BOUND ( 'NONE', #125938, .T. ) ;
#30100=ORIENTED_EDGE ( 'NONE', *, *, #94914, .F. ) ;
#30101=EDGE_LOOP ( 'NONE', ( #82139, #96495, #50346, #87342 ) ) ;
#30102=CARTESIAN_POINT ( 'NONE',  ( -11.64999999999999680, 2.500000000000000000, 1.472243186433545459 ) ) ;
#30103=CIRCLE ( 'NONE', #90719, 0.1000000000000000472 ) ;
#30104=CONICAL_SURFACE ( 'NONE', #28028, 0.1000000000000000472, 0.003490658503988666988 ) ;
#30105=CARTESIAN_POINT ( 'NONE',  ( -15.19999999999998330, 2.500000000000000000, 0.3464101615137758494 ) ) ;
#30106=FACE_BOUND ( 'NONE', #91610, .T. ) ;
#30107=DIRECTION ( 'NONE',  ( 0.000000000000000000, 0.000000000000000000, 1.000000000000000000 ) ) ;
#30108=DIRECTION ( 'NONE',  ( -0.000000000000000000, -1.000000000000000000, -0.000000000000000000 ) ) ;
#30109=DIRECTION ( 'NONE',  ( 0.000000000000000000, -0.9999939076577903929, 0.003490651415223739937 ) ) ;
#30110=CONICAL_SURFACE ( 'NONE', #48978, 0.1000000000000002554, 0.003490658503988666988 ) ;
#30111=CONICAL_SURFACE ( 'NONE', #55229, 0.1000000000000002554, 0.003490658503988666988 ) ;
#30112=AXIS2_PLACEMENT_3D ( 'NONE', #103739, #117227, #104372 ) ;
#30113=CARTESIAN_POINT ( 'NONE',  ( -1.850000000000033396, 2.500000000000000000, -6.841600689897077814 ) ) ;
#30114=DIRECTION ( 'NONE',  ( 0.000000000000000000, 1.000000000000000000, 0.000000000000000000 ) ) ;
#30115=FACE_OUTER_BOUND ( 'NONE', #66438, .T. ) ;
#30116=DIRECTION ( 'NONE',  ( 0.000000000000000000, 1.000000000000000000, 0.000000000000000000 ) ) ;
#30117=ORIENTED_EDGE ( 'NONE', *, *, #78204, .T. ) ;
#30118=CIRCLE ( 'NONE', #11317, 0.1000000000000002554 ) ;
#30119=DIRECTION ( 'NONE',  ( 0.000000000000000000, 0.000000000000000000, -1.000000000000000000 ) ) ;
#30120=CIRCLE ( 'NONE', #7089, 0.1000000000000000472 ) ;
#30121=CARTESIAN_POINT ( 'NONE',  ( 9.199999999999915801, 12.50000000000000000, 4.395220292106234439 ) ) ;
#30122=ORIENTED_EDGE ( 'NONE', *, *, #35822, .T. ) ;
#30123=EDGE_LOOP ( 'NONE', ( #101261, #68354, #95075, #115971 ) ) ;
#30124=DIRECTION ( 'NONE',  ( 0.000000000000000000, -0.9999939076577903929, 0.003490651415223739937 ) ) ;
#30125=CARTESIAN_POINT ( 'NONE',  ( 4.399999999999940847, 2.500000000000000000, -4.676537180435977881 ) ) ;
#30126=FACE_BOUND ( 'NONE', #116902, .T. ) ;
#30127=DIRECTION ( 'NONE',  ( 0.000000000000000000, 0.000000000000000000, 1.000000000000000000 ) ) ;
#30128=EDGE_CURVE ( 'NONE', #64157, #11947, #55333, .T. ) ;
#30129=FACE_OUTER_BOUND ( 'NONE', #100080, .T. ) ;
#30130=ADVANCED_FACE ( 'NONE', ( #65925 ), #97183, .T. ) ;
#30131=VERTEX_POINT ( 'NONE', #17459 ) ;
#30132=DIRECTION ( 'NONE',  ( -0.000000000000000000, 1.000000000000000000, -0.000000000000000000 ) ) ;
#30133=CARTESIAN_POINT ( 'NONE',  ( -14.14999999999998614, 12.50000000000000000, -2.165063509461099489 ) ) ;
#30134=VECTOR ( 'NONE', #97959, 1000.000000000000000 ) ;
#30135=ORIENTED_EDGE ( 'NONE', *, *, #36103, .F. ) ;
#30136=CARTESIAN_POINT ( 'NONE',  ( 10.59999999999991260, 2.500000000000000000, 0.3464101615137735735 ) ) ;
#30137=LINE ( 'NONE', #38673, #107601 ) ;
#30138=EDGE_CURVE ( 'NONE', #101406, #123848, #17658, .T. ) ;
#30139=DIRECTION ( 'NONE',  ( 0.000000000000000000, 1.000000000000000000, 0.000000000000000000 ) ) ;
#30140=FACE_OUTER_BOUND ( 'NONE', #10098, .T. ) ;
#30141=CIRCLE ( 'NONE', #80310, 0.06509327318403745899 ) ;
#30142=AXIS2_PLACEMENT_3D ( 'NONE', #106705, #127017, #7210 ) ;
#30143=ORIENTED_EDGE ( 'NONE', *, *, #22360, .F. ) ;
#30144=DIRECTION ( 'NONE',  ( 0.000000000000000000, 0.000000000000000000, 1.000000000000000000 ) ) ;
#30145=DIRECTION ( 'NONE',  ( -4.274815082592931898E-19, -0.9999939076577903929, -0.003490651415223739937 ) ) ;
#30146=CARTESIAN_POINT ( 'NONE',  ( -11.89999999999999680, 12.50000000000000000, -3.983716857408423628 ) ) ;
#30147=DIRECTION ( 'NONE',  ( 0.000000000000000000, 1.000000000000000000, 0.000000000000000000 ) ) ;
#30148=ORIENTED_EDGE ( 'NONE', *, *, #7883, .T. ) ;
#30149=ORIENTED_EDGE ( 'NONE', *, *, #53412, .T. ) ;
#30150=CIRCLE ( 'NONE', #69848, 0.1000000000000000472 ) ;
#30151=CARTESIAN_POINT ( 'NONE',  ( 4.599999999999935696, 12.50000000000000000, 4.957854068765711553 ) ) ;
#30152=EDGE_LOOP ( 'NONE', ( #19336, #90316, #97575, #40216 ) ) ;
#30153=DIRECTION ( 'NONE',  ( 0.000000000000000000, 1.000000000000000000, 0.000000000000000000 ) ) ;
#30154=DIRECTION ( 'NONE',  ( -0.000000000000000000, 1.000000000000000000, -0.000000000000000000 ) ) ;
#30155=DIRECTION ( 'NONE',  ( 0.000000000000000000, 1.000000000000000000, 0.000000000000000000 ) ) ;
#30156=ORIENTED_EDGE ( 'NONE', *, *, #82059, .T. ) ;
#30157=DIRECTION ( 'NONE',  ( 0.000000000000000000, 0.000000000000000000, 1.000000000000000000 ) ) ;
#30158=DIRECTION ( 'NONE',  ( -0.000000000000000000, -1.000000000000000000, -0.000000000000000000 ) ) ;
#30159=DIRECTION ( 'NONE',  ( -0.000000000000000000, -1.000000000000000000, -0.000000000000000000 ) ) ;
#30160=LINE ( 'NONE', #41273, #101960 ) ;
#30161=CARTESIAN_POINT ( 'NONE',  ( 4.399999999999937295, 12.50000000000000000, 4.741630453620009789 ) ) ;
#30162=CARTESIAN_POINT ( 'NONE',  ( -1.050000000000037348, 12.50000000000000000, -2.511473670974877948 ) ) ;
#30163=EDGE_LOOP ( 'NONE', ( #83607, #39768, #120313, #25812 ) ) ;
#30164=EDGE_LOOP ( 'NONE', ( #91439, #96464 ) ) ;
#30165=DIRECTION ( 'NONE',  ( 0.000000000000000000, 0.000000000000000000, 1.000000000000000000 ) ) ;
#30166=AXIS2_PLACEMENT_3D ( 'NONE', #53754, #123765, #64214 ) ;
#30167=ORIENTED_EDGE ( 'NONE', *, *, #75454, .T. ) ;
#30168=AXIS2_PLACEMENT_3D ( 'NONE', #93553, #111909, #123637 ) ;
#30169=CIRCLE ( 'NONE', #36431, 0.1000000000000002554 ) ;
#30171=ORIENTED_EDGE ( 'NONE', *, *, #98939, .F. ) ;
#30172=ORIENTED_EDGE ( 'NONE', *, *, #117636, .T. ) ;
#30173=ORIENTED_EDGE ( 'NONE', *, *, #82868, .T. ) ;
#30174=VECTOR ( 'NONE', #91781, 1000.000000000000000 ) ;
#30175=CARTESIAN_POINT ( 'NONE',  ( -2.900000000000029665, 2.500000000000000000, 3.537306695894645081 ) ) ;
#30176=AXIS2_PLACEMENT_3D ( 'NONE', #9649, #98656, #8349 ) ;
#30177=CARTESIAN_POINT ( 'NONE',  ( -13.74999999999995381, 2.500000000000000000, -2.065063509461099844 ) ) ;
#30178=CARTESIAN_POINT ( 'NONE',  ( -2.900000000000029665, 2.500000000000000000, 3.737306695894644371 ) ) ;
#30180=DIRECTION ( 'NONE',  ( -0.000000000000000000, 1.000000000000000000, -0.000000000000000000 ) ) ;
#30181=CARTESIAN_POINT ( 'NONE',  ( 4.799999999999939426, 2.500000000000000000, -4.676537180435977881 ) ) ;
#30183=EDGE_CURVE ( 'NONE', #32860, #105669, #126444, .T. ) ;
#30184=DIRECTION ( 'NONE',  ( 0.000000000000000000, 0.000000000000000000, 1.000000000000000000 ) ) ;
#30185=FACE_OUTER_BOUND ( 'NONE', #122213, .T. ) ;
#30186=ADVANCED_FACE ( 'NONE', ( #105209 ), #126141, .T. ) ;
#30187=DIRECTION ( 'NONE',  ( -4.274815082592931898E-19, -0.9999939076577903929, -0.003490651415223739937 ) ) ;
#30190=AXIS2_PLACEMENT_3D ( 'NONE', #85079, #62870, #102771 ) ;
#30191=AXIS2_PLACEMENT_3D ( 'NONE', #93459, #122928, #103925 ) ;
#30192=FACE_OUTER_BOUND ( 'NONE', #79337, .T. ) ;
#30193=CIRCLE ( 'NONE', #105391, 0.06509327318403745899 ) ;
#30194=CIRCLE ( 'NONE', #103345, 0.1000000000000002554 ) ;
#30195=ORIENTED_EDGE ( 'NONE', *, *, #115017, .F. ) ;
#30196=ADVANCED_FACE ( 'NONE', ( #128083 ), #74121, .T. ) ;
#30197=EDGE_LOOP ( 'NONE', ( #93434, #76114, #29290, #121534 ) ) ;
#30198=DIRECTION ( 'NONE',  ( -4.274815082592931898E-19, -0.9999939076577903929, -0.003490651415223739937 ) ) ;
#30199=CARTESIAN_POINT ( 'NONE',  ( 8.099999999999923261, 12.50000000000000000, 4.611443907251934426 ) ) ;
#30200=AXIS2_PLACEMENT_3D ( 'NONE', #127168, #8013, #6071 ) ;
#30201=CIRCLE ( 'NONE', #92978, 0.06509327318403745899 ) ;
#30202=DIRECTION ( 'NONE',  ( 0.000000000000000000, 0.000000000000000000, -1.000000000000000000 ) ) ;
#30203=CIRCLE ( 'NONE', #67829, 0.06509327318403741736 ) ;
#30204=DIRECTION ( 'NONE',  ( 0.000000000000000000, -0.000000000000000000, 1.000000000000000000 ) ) ;
#30205=CARTESIAN_POINT ( 'NONE',  ( 8.949999999999917577, 2.500000000000000000, 6.248780366869520542 ) ) ;
#30206=DIRECTION ( 'NONE',  ( 0.000000000000000000, -0.000000000000000000, 1.000000000000000000 ) ) ;
#30208=CONICAL_SURFACE ( 'NONE', #119783, 0.09999999999999999167, 0.003490658503988666988 ) ;
#30209=CIRCLE ( 'NONE', #46932, 0.1000000000000002554 ) ;
#30210=VERTEX_POINT ( 'NONE', #67185 ) ;
#30211=CARTESIAN_POINT ( 'NONE',  ( 11.64999999999990798, 12.50000000000000000, -2.922977105672691422 ) ) ;
#30212=AXIS2_PLACEMENT_3D ( 'NONE', #4487, #54900, #66015 ) ;
#30213=ORIENTED_EDGE ( 'NONE', *, *, #99226, .T. ) ;
#30214=DIRECTION ( 'NONE',  ( 0.000000000000000000, -0.000000000000000000, 1.000000000000000000 ) ) ;
#30215=EDGE_CURVE ( 'NONE', #72305, #110447, #37132, .T. ) ;
#30216=EDGE_LOOP ( 'NONE', ( #46683, #105900 ) ) ;
#30217=AXIS2_PLACEMENT_3D ( 'NONE', #53547, #24085, #72550 ) ;
#30218=ORIENTED_EDGE ( 'NONE', *, *, #94480, .T. ) ;
#30219=CARTESIAN_POINT ( 'NONE',  ( 8.149999999999920419, 2.500000000000000000, -2.411473670974877859 ) ) ;
#30220=CARTESIAN_POINT ( 'NONE',  ( -8.950000000000009948, 2.500000000000000000, -1.818653347947326138 ) ) ;
#30221=EDGE_CURVE ( 'NONE', #119823, #63624, #90828, .T. ) ;
#30222=DIRECTION ( 'NONE',  ( 0.000000000000000000, 1.000000000000000000, 0.000000000000000000 ) ) ;
#30223=FACE_OUTER_BOUND ( 'NONE', #14345, .T. ) ;
#30224=DIRECTION ( 'NONE',  ( -0.000000000000000000, -1.000000000000000000, -0.000000000000000000 ) ) ;
#30225=VERTEX_POINT ( 'NONE', #117581 ) ;
#30226=DIRECTION ( 'NONE',  ( 0.000000000000000000, 0.000000000000000000, -1.000000000000000000 ) ) ;
#30227=CARTESIAN_POINT ( 'NONE',  ( -7.950000000000016165, 12.50000000000000000, -6.495190528383297135 ) ) ;
#30228=EDGE_CURVE ( 'NONE', #96489, #39393, #103453, .T. ) ;
#30229=EDGE_CURVE ( 'NONE', #67757, #21708, #107560, .T. ) ;
#30230=FACE_OUTER_BOUND ( 'NONE', #28745, .T. ) ;
#30231=EDGE_CURVE ( 'NONE', #119121, #124307, #51141, .T. ) ;
#30232=PLANE ( 'NONE',  #36812 ) ;
#30233=ADVANCED_FACE ( 'NONE', ( #56726 ), #88781, .T. ) ;
#30234=AXIS2_PLACEMENT_3D ( 'NONE', #88790, #21331, #389 ) ;
#30235=FACE_OUTER_BOUND ( 'NONE', #54012, .T. ) ;
#30236=ORIENTED_EDGE ( 'NONE', *, *, #128872, .F. ) ;
#30237=VERTEX_POINT ( 'NONE', #56101 ) ;
#30238=EDGE_CURVE ( 'NONE', #7578, #53869, #8290, .T. ) ;
#30239=DIRECTION ( 'NONE',  ( 0.000000000000000000, 1.000000000000000000, 0.000000000000000000 ) ) ;
#30240=EDGE_CURVE ( 'NONE', #120360, #96594, #45662, .T. ) ;
#30241=VERTEX_POINT ( 'NONE', #85572 ) ;
#30242=AXIS2_PLACEMENT_3D ( 'NONE', #61362, #13528, #53477 ) ;
#30243=CARTESIAN_POINT ( 'NONE',  ( 1.449999999999952216, 12.50000000000000000, 1.753560074763284016 ) ) ;
#30244=DIRECTION ( 'NONE',  ( -0.000000000000000000, 1.000000000000000000, -0.000000000000000000 ) ) ;
#30245=AXIS2_PLACEMENT_3D ( 'NONE', #8499, #30116, #28818 ) ;
#30246=ADVANCED_FACE ( 'NONE', ( #96039 ), #125493, .T. ) ;
#30247=B_SPLINE_CURVE_WITH_KNOTS ( 'NONE', 3,
 ( #45517, #85422, #97179, #25866, #126648, #46142, #65775, #38269 ),
 .UNSPECIFIED., .F., .F.,
 ( 4, 2, 2, 4 ),
 ( 0.000000000000000000, 0.01659299152883686457, 0.03318598305767372914, 0.06637196611534749990 ),
 .UNSPECIFIED. ) ;
#30248=ORIENTED_EDGE ( 'NONE', *, *, #46428, .F. ) ;
#30249=DIRECTION ( 'NONE',  ( 0.000000000000000000, 1.000000000000000000, 0.000000000000000000 ) ) ;
#30250=DIRECTION ( 'NONE',  ( -0.000000000000000000, 1.000000000000000000, -0.000000000000000000 ) ) ;
#30251=EDGE_CURVE ( 'NONE', #103678, #41488, #111765, .T. ) ;
#30253=CARTESIAN_POINT ( 'NONE',  ( 1.249999999999952482, 12.50000000000000000, -5.802370205355749988 ) ) ;
#30254=EDGE_CURVE ( 'NONE', #40749, #50291, #15601, .T. ) ;
#30255=CONICAL_SURFACE ( 'NONE', #103395, 0.1000000000000000472, 0.003490658503988666988 ) ;
#30256=FACE_OUTER_BOUND ( 'NONE', #91066, .T. ) ;
#30257=CIRCLE ( 'NONE', #67875, 0.06509327318403745899 ) ;
#30258=EDGE_LOOP ( 'NONE', ( #93867, #102590 ) ) ;
#30259=CARTESIAN_POINT ( 'NONE',  ( 6.649999999999929301, 12.50000000000000000, 6.495190528383297135 ) ) ;
#30260=CARTESIAN_POINT ( 'NONE',  ( 9.149999999999916866, 2.500000000000000000, 7.288010851410849256 ) ) ;
#30261=CARTESIAN_POINT ( 'NONE',  ( 13.34999999999989662, 12.50000000000000000, -1.472243186433550122 ) ) ;
#30262=ORIENTED_EDGE ( 'NONE', *, *, #9782, .F. ) ;
#30263=AXIS2_PLACEMENT_3D ( 'NONE', #20640, #47519, #7567 ) ;
#30264=AXIS2_PLACEMENT_3D ( 'NONE', #71489, #111402, #21762 ) ;
#30265=VERTEX_POINT ( 'NONE', #21338 ) ;
#30266=DIRECTION ( 'NONE',  ( 0.000000000000000000, -0.9999939076577903929, 0.003490651415223739937 ) ) ;
#30267=DIRECTION ( 'NONE',  ( 0.000000000000000000, 0.000000000000000000, 1.000000000000000000 ) ) ;
#30268=DIRECTION ( 'NONE',  ( -0.000000000000000000, -1.000000000000000000, -0.000000000000000000 ) ) ;
#30269=AXIS2_PLACEMENT_3D ( 'NONE', #105765, #76305, #4307 ) ;
#30270=ORIENTED_EDGE ( 'NONE', *, *, #4668, .T. ) ;
#30271=DIRECTION ( 'NONE',  ( -0.000000000000000000, 1.000000000000000000, -0.000000000000000000 ) ) ;
#30272=CARTESIAN_POINT ( 'NONE',  ( -7.700000000000012612, 12.50000000000000000, 4.676537180435972552 ) ) ;
#30273=ORIENTED_EDGE ( 'NONE', *, *, #34631, .F. ) ;
#30274=DIRECTION ( 'NONE',  ( 0.000000000000000000, 0.000000000000000000, 1.000000000000000000 ) ) ;
#30275=VERTEX_POINT ( 'NONE', #70450 ) ;
#30276=DIRECTION ( 'NONE',  ( 0.000000000000000000, 0.000000000000000000, 1.000000000000000000 ) ) ;
#30277=EDGE_CURVE ( 'NONE', #73222, #65306, #118254, .T. ) ;
#30278=CIRCLE ( 'NONE', #65941, 0.06509327318403741736 ) ;
#30279=ORIENTED_EDGE ( 'NONE', *, *, #83709, .F. ) ;
#30280=DIRECTION ( 'NONE',  ( 0.000000000000000000, 0.000000000000000000, -1.000000000000000000 ) ) ;
#30281=CARTESIAN_POINT ( 'NONE',  ( 13.92826131978669046, 2.499999999999999112, -6.790916465128549184 ) ) ;
#30282=AXIS2_PLACEMENT_3D ( 'NONE', #72393, #21335, #80913 ) ;
#30283=EDGE_CURVE ( 'NONE', #117070, #55871, #20070, .T. ) ;
#30284=AXIS2_PLACEMENT_3D ( 'NONE', #124690, #35036, #25839 ) ;
#30285=AXIS2_PLACEMENT_3D ( 'NONE', #88063, #7592, #116891 ) ;
#30286=ORIENTED_EDGE ( 'NONE', *, *, #25110, .T. ) ;
#30287=EDGE_LOOP ( 'NONE', ( #93962, #97155, #93527, #41101 ) ) ;
#30288=DIRECTION ( 'NONE',  ( 0.000000000000000000, 0.000000000000000000, 1.000000000000000000 ) ) ;
#30289=DIRECTION ( 'NONE',  ( 0.000000000000000000, -0.9999939076577903929, 0.003490651415223739937 ) ) ;
#30290=ORIENTED_EDGE ( 'NONE', *, *, #16879, .T. ) ;
#30291=PLANE ( 'NONE',  #40596 ) ;
#30293=CIRCLE ( 'NONE', #55406, 0.06509327318403745899 ) ;
#30294=AXIS2_PLACEMENT_3D ( 'NONE', #68973, #119356, #116776 ) ;
#30295=PLANE ( 'NONE',  #22340 ) ;
#30297=CARTESIAN_POINT ( 'NONE',  ( 11.44999999999991047, 2.500000000000000000, 6.248780366869520542 ) ) ;
#30298=AXIS2_PLACEMENT_3D ( 'NONE', #8947, #120214, #111684 ) ;
#30299=CARTESIAN_POINT ( 'NONE',  ( 11.24999999999991118, 2.500000000000000000, 5.902370205355745192 ) ) ;
#30300=DIRECTION ( 'NONE',  ( -0.000000000000000000, -1.000000000000000000, -0.000000000000000000 ) ) ;
#30301=AXIS2_PLACEMENT_3D ( 'NONE', #26012, #94099, #55467 ) ;
#30302=AXIS2_PLACEMENT_3D ( 'NONE', #84368, #26105, #104640 ) ;
#30303=ORIENTED_EDGE ( 'NONE', *, *, #128158, .T. ) ;
#30304=ORIENTED_EDGE ( 'NONE', *, *, #38584, .T. ) ;
#30305=VERTEX_POINT ( 'NONE', #30547 ) ;
#30306=DIRECTION ( 'NONE',  ( 0.000000000000000000, -0.9999939076577903929, 0.003490651415223739937 ) ) ;
#30307=DIRECTION ( 'NONE',  ( 0.000000000000000000, 1.000000000000000000, 0.000000000000000000 ) ) ;
#30308=AXIS2_PLACEMENT_3D ( 'NONE', #57409, #86857, #26660 ) ;
#30309=DIRECTION ( 'NONE',  ( 0.000000000000000000, 0.000000000000000000, -1.000000000000000000 ) ) ;
#30310=ORIENTED_EDGE ( 'NONE', *, *, #119539, .F. ) ;
#30312=FACE_BOUND ( 'NONE', #100347, .T. ) ;
#30313=ORIENTED_EDGE ( 'NONE', *, *, #15548, .T. ) ;
#30314=DIRECTION ( 'NONE',  ( 0.000000000000000000, 0.000000000000000000, -1.000000000000000000 ) ) ;
#30315=DIRECTION ( 'NONE',  ( -0.000000000000000000, 1.000000000000000000, -0.000000000000000000 ) ) ;
#30316=CARTESIAN_POINT ( 'NONE',  ( -11.04999999999999893, 2.500000000000000000, 1.918653347947321564 ) ) ;
#30317=FACE_OUTER_BOUND ( 'NONE', #43174, .T. ) ;
#30318=DIRECTION ( 'NONE',  ( 0.000000000000000000, 0.000000000000000000, -1.000000000000000000 ) ) ;
#30320=PLANE ( 'NONE',  #127881 ) ;
#30321=LINE ( 'NONE', #67631, #114287 ) ;
#30322=CONICAL_SURFACE ( 'NONE', #49200, 0.1000000000000000472, 0.003490658503988666988 ) ;
#30323=DIRECTION ( 'NONE',  ( -0.000000000000000000, -1.000000000000000000, -0.000000000000000000 ) ) ;
#30324=ADVANCED_FACE ( 'NONE', ( #79620 ), #69142, .T. ) ;
#30326=ORIENTED_EDGE ( 'NONE', *, *, #62660, .F. ) ;
#30327=ORIENTED_EDGE ( 'NONE', *, *, #118802, .F. ) ;
#30328=ORIENTED_EDGE ( 'NONE', *, *, #49578, .F. ) ;
#30329=CARTESIAN_POINT ( 'NONE',  ( -2.900000000000029221, 2.500000000000000000, -5.022947341949754119 ) ) ;
#30330=DIRECTION ( 'NONE',  ( 0.000000000000000000, 0.000000000000000000, -1.000000000000000000 ) ) ;
#30331=ORIENTED_EDGE ( 'NONE', *, *, #73035, .F. ) ;
#30332=VERTEX_POINT ( 'NONE', #8927 ) ;
#30333=ORIENTED_EDGE ( 'NONE', *, *, #110564, .F. ) ;
#30334=DIRECTION ( 'NONE',  ( 0.000000000000000000, 1.000000000000000000, 0.000000000000000000 ) ) ;
#30335=CONICAL_SURFACE ( 'NONE', #3128, 0.1000000000000002554, 0.003490658503988666988 ) ;
#30336=EDGE_CURVE ( 'NONE', #22266, #79729, #19829, .T. ) ;
#30337=CIRCLE ( 'NONE', #101420, 0.06509327318403745899 ) ;
#30338=DIRECTION ( 'NONE',  ( 0.000000000000000000, 0.000000000000000000, 1.000000000000000000 ) ) ;
#30339=DIRECTION ( 'NONE',  ( 0.000000000000000000, 1.000000000000000000, 0.000000000000000000 ) ) ;
#30340=CARTESIAN_POINT ( 'NONE',  ( -5.650000000000023448, 12.50000000000000000, -6.841600689897078702 ) ) ;
#30341=DIRECTION ( 'NONE',  ( 0.000000000000000000, 0.000000000000000000, -1.000000000000000000 ) ) ;
#30342=DIRECTION ( 'NONE',  ( 0.000000000000000000, 1.000000000000000000, 0.000000000000000000 ) ) ;
#30343=EDGE_CURVE ( 'NONE', #53599, #72890, #82533, .T. ) ;
#30344=CARTESIAN_POINT ( 'NONE',  ( -12.09999999999999609, 2.500000000000000000, 0.1000000000000017403 ) ) ;
#30345=ADVANCED_FACE ( 'NONE', ( #100541 ), #99915, .T. ) ;
#30346=ORIENTED_EDGE ( 'NONE', *, *, #18974, .T. ) ;
#30347=CARTESIAN_POINT ( 'NONE',  ( -0.4000000000000331624, 2.500000000000000000, 0.000000000000000000 ) ) ;
#30348=ORIENTED_EDGE ( 'NONE', *, *, #75302, .F. ) ;
#30349=CIRCLE ( 'NONE', #122276, 0.06509327318403745899 ) ;
#30350=ORIENTED_EDGE ( 'NONE', *, *, #33319, .T. ) ;
#30351=VERTEX_POINT ( 'NONE', #29880 ) ;
#30352=AXIS2_PLACEMENT_3D ( 'NONE', #47681, #87581, #8375 ) ;
#30353=CARTESIAN_POINT ( 'NONE',  ( 11.44999999999990692, 2.500000000000000000, 1.918653347947321564 ) ) ;
#30354=ORIENTED_EDGE ( 'NONE', *, *, #63590, .F. ) ;
#30355=EDGE_CURVE ( 'NONE', #15089, #52919, #99259, .T. ) ;
#30356=ORIENTED_EDGE ( 'NONE', *, *, #55131, .T. ) ;
#30357=CARTESIAN_POINT ( 'NONE',  ( -8.550000000000011369, 2.500000000000000000, 1.918653347947321564 ) ) ;
#30358=DIRECTION ( 'NONE',  ( 0.000000000000000000, 0.000000000000000000, 1.000000000000000000 ) ) ;
#30360=CIRCLE ( 'NONE', #26138, 0.06509327318403745899 ) ;
#30361=FACE_OUTER_BOUND ( 'NONE', #88206, .T. ) ;
#30362=DIRECTION ( 'NONE',  ( -0.000000000000000000, -1.000000000000000000, -0.000000000000000000 ) ) ;
#30363=VERTEX_POINT ( 'NONE', #119533 ) ;
#30364=CARTESIAN_POINT ( 'NONE',  ( -14.14999999999998792, 2.500000000000000000, 2.857883832488652853 ) ) ;
#30365=ORIENTED_EDGE ( 'NONE', *, *, #16884, .F. ) ;
#30366=DIRECTION ( 'NONE',  ( 0.000000000000000000, 1.000000000000000000, 0.000000000000000000 ) ) ;
#30367=EDGE_LOOP ( 'NONE', ( #105560, #53504 ) ) ;
#30368=CARTESIAN_POINT ( 'NONE',  ( 2.949999999999946887, 2.500000000000000000, -6.495190528383302464 ) ) ;
#30369=DIRECTION ( 'NONE',  ( 0.000000000000000000, 1.000000000000000000, 0.000000000000000000 ) ) ;
#30370=ORIENTED_EDGE ( 'NONE', *, *, #79852, .F. ) ;
#30371=DIRECTION ( 'NONE',  ( -0.000000000000000000, -1.000000000000000000, -0.000000000000000000 ) ) ;
#30372=DIRECTION ( 'NONE',  ( 0.000000000000000000, 0.000000000000000000, 1.000000000000000000 ) ) ;
#30373=VERTEX_POINT ( 'NONE', #80275 ) ;
#30374=EDGE_CURVE ( 'NONE', #56130, #93025, #108428, .T. ) ;
#30375=VECTOR ( 'NONE', #60577, 1000.000000000000000 ) ;
#30376=AXIS2_PLACEMENT_3D ( 'NONE', #52098, #92015, #63201 ) ;
#30377=PLANE ( 'NONE',  #32073 ) ;
#30378=ORIENTED_EDGE ( 'NONE', *, *, #39680, .T. ) ;
#30379=AXIS2_PLACEMENT_3D ( 'NONE', #125135, #35472, #75370 ) ;
#30380=EDGE_LOOP ( 'NONE', ( #54694, #14576 ) ) ;
#30381=CARTESIAN_POINT ( 'NONE',  ( 1.049999999999954969, 12.50000000000000000, -6.776507416713039689 ) ) ;
#30382=DIRECTION ( 'NONE',  ( 0.000000000000000000, 0.000000000000000000, -1.000000000000000000 ) ) ;
#30383=ADVANCED_FACE ( 'NONE', ( #50181 ), #3106, .T. ) ;
#30385=CARTESIAN_POINT ( 'NONE',  ( -11.25000000000000000, 2.500000000000000000, -7.288010851410851032 ) ) ;
#30386=EDGE_CURVE ( 'NONE', #116756, #37559, #44878, .T. ) ;
#30387=CIRCLE ( 'NONE', #15770, 0.1000000000000000472 ) ;
#30388=CARTESIAN_POINT ( 'NONE',  ( 9.399999999999918643, 2.500000000000000000, -0.4464101615137782142 ) ) ;
#30389=AXIS2_PLACEMENT_3D ( 'NONE', #22121, #42388, #82317 ) ;
#30390=ORIENTED_EDGE ( 'NONE', *, *, #118706, .F. ) ;
#30392=FACE_OUTER_BOUND ( 'NONE', #98259, .T. ) ;
#30393=EDGE_CURVE ( 'NONE', #51160, #81889, #21993, .T. ) ;
#30394=CIRCLE ( 'NONE', #47113, 0.1000000000000000472 ) ;
#30395=ADVANCED_FACE ( 'NONE', ( #48892 ), #128609, .T. ) ;
#30396=EDGE_CURVE ( 'NONE', #73228, #59490, #38730, .T. ) ;
#30397=ADVANCED_FACE ( 'NONE', ( #39080 ), #78996, .T. ) ;
#30398=ORIENTED_EDGE ( 'NONE', *, *, #13330, .T. ) ;
#30399=CONICAL_SURFACE ( 'NONE', #1119, 0.1000000000000002554, 0.003490658503988666988 ) ;
#30400=DIRECTION ( 'NONE',  ( 0.000000000000000000, 0.000000000000000000, 1.000000000000000000 ) ) ;
#30401=CARTESIAN_POINT ( 'NONE',  ( -4.550000000000026468, 2.500000000000000000, -6.495190528383302464 ) ) ;
#30402=AXIS2_PLACEMENT_3D ( 'NONE', #14009, #4185, #83426 ) ;
#30403=EDGE_CURVE ( 'NONE', #28942, #125792, #99275, .T. ) ;
#30404=AXIS2_PLACEMENT_3D ( 'NONE', #6655, #39408, #109400 ) ;
#30406=LINE ( 'NONE', #2848, #69896 ) ;
#30407=FACE_OUTER_BOUND ( 'NONE', #91566, .T. ) ;
#30408=DIRECTION ( 'NONE',  ( -0.000000000000000000, -1.000000000000000000, -0.000000000000000000 ) ) ;
#30409=CARTESIAN_POINT ( 'NONE',  ( -0.8500000000000382805, 12.50000000000000000, -5.802370205355749988 ) ) ;
#30410=ORIENTED_EDGE ( 'NONE', *, *, #65949, .F. ) ;
#30411=EDGE_CURVE ( 'NONE', #112989, #25435, #89442, .T. ) ;
#30412=DIRECTION ( 'NONE',  ( 0.000000000000000000, 1.000000000000000000, 0.000000000000000000 ) ) ;
#30413=CARTESIAN_POINT ( 'NONE',  ( -5.850000000000021849, 2.500000000000000000, -7.288010851410854585 ) ) ;
#30414=DIRECTION ( 'NONE',  ( -0.000000000000000000, 1.000000000000000000, -0.000000000000000000 ) ) ;
#30415=AXIS2_PLACEMENT_3D ( 'NONE', #72792, #112718, #123799 ) ;
#30416=ORIENTED_EDGE ( 'NONE', *, *, #80193, .T. ) ;
#30417=DIRECTION ( 'NONE',  ( 0.000000000000000000, 0.000000000000000000, 1.000000000000000000 ) ) ;
#30418=ORIENTED_EDGE ( 'NONE', *, *, #52848, .F. ) ;
#30419=EDGE_LOOP ( 'NONE', ( #109081, #125694 ) ) ;
#30420=DIRECTION ( 'NONE',  ( -0.000000000000000000, 1.000000000000000000, -0.000000000000000000 ) ) ;
#30421=VECTOR ( 'NONE', #15130, 1000.000000000000000 ) ;
#30422=ORIENTED_EDGE ( 'NONE', *, *, #104583, .F. ) ;
#30423=B_SPLINE_CURVE_WITH_KNOTS ( 'NONE', 3,
 ( #87083, #117171, #17022, #56972, #7882, #96908, #27508, #47835, #67420, #107381, #17698, #122370 ),
 .UNSPECIFIED., .F., .F.,
 ( 4, 2, 2, 2, 2, 4 ),
 ( 4.337147489887063328E-18, 0.0006571239767409316418, 0.001314247953481858947, 0.002628495906963720496, 0.003942743860445582262, 0.005256991813927443594 ),
 .UNSPECIFIED. ) ;
#30424=CARTESIAN_POINT ( 'NONE',  ( 11.69999999999990870, 2.500000000000000000, -4.330127018922201643 ) ) ;
#30425=CARTESIAN_POINT ( 'NONE',  ( -10.00000000000000533, 2.500000000000000000, 0.6928203230275494784 ) ) ;
#30426=CONICAL_SURFACE ( 'NONE', #34725, 0.1000000000000002554, 0.003490658503988666988 ) ;
#30427=AXIS2_PLACEMENT_3D ( 'NONE', #69059, #67771, #28505 ) ;
#30428=ORIENTED_EDGE ( 'NONE', *, *, #115736, .T. ) ;
#30429=CARTESIAN_POINT ( 'NONE',  ( 4.999999999999936939, 2.500000000000000000, -0.6928203230275541413 ) ) ;
#30430=DIRECTION ( 'NONE',  ( -0.000000000000000000, -1.000000000000000000, -0.000000000000000000 ) ) ;
#30431=CARTESIAN_POINT ( 'NONE',  ( 16.32360635137687410, -2.500000000000000000, -4.874197684290930255 ) ) ;
#30433=ORIENTED_EDGE ( 'NONE', *, *, #35685, .T. ) ;
#30434=VECTOR ( 'NONE', #24283, 1000.000000000000000 ) ;
#30435=EDGE_CURVE ( 'NONE', #84709, #103499, #14568, .T. ) ;
#30436=ORIENTED_EDGE ( 'NONE', *, *, #31185, .T. ) ;
#30437=CIRCLE ( 'NONE', #105640, 0.06509327318403745899 ) ;
#30438=ORIENTED_EDGE ( 'NONE', *, *, #55722, .F. ) ;
#30439=DIRECTION ( 'NONE',  ( 0.000000000000000000, 0.000000000000000000, 1.000000000000000000 ) ) ;
#30440=PLANE ( 'NONE',  #66684 ) ;
#30441=CARTESIAN_POINT ( 'NONE',  ( -11.64999999999999858, 2.500000000000000000, -1.472243186433546125 ) ) ;
#30442=FACE_BOUND ( 'NONE', #76001, .T. ) ;
#30443=EDGE_LOOP ( 'NONE', ( #44008, #5348 ) ) ;
#30444=DIRECTION ( 'NONE',  ( -0.000000000000000000, 1.000000000000000000, -0.000000000000000000 ) ) ;
#30445=DIRECTION ( 'NONE',  ( 0.000000000000000000, 0.000000000000000000, 1.000000000000000000 ) ) ;
#30446=ORIENTED_EDGE ( 'NONE', *, *, #42899, .T. ) ;
#30447=EDGE_CURVE ( 'NONE', #51458, #30363, #109803, .T. ) ;
#30448=DIRECTION ( 'NONE',  ( -0.7336674352945157240, 0.000000000000000000, 0.6795087154616692438 ) ) ;
#30449=AXIS2_PLACEMENT_3D ( 'NONE', #13185, #105459, #125714 ) ;
#30450=CARTESIAN_POINT ( 'NONE',  ( -11.69999999999999929, 2.500000000000000000, -0.09999999999999827083 ) ) ;
#30451=AXIS2_PLACEMENT_3D ( 'NONE', #27077, #58488, #78112 ) ;
#30452=CARTESIAN_POINT ( 'NONE',  ( 5.849999999999934808, 2.500000000000000000, -5.902370205355750521 ) ) ;
#30453=DIRECTION ( 'NONE',  ( 0.000000000000000000, 1.000000000000000000, 0.000000000000000000 ) ) ;
#30454=CARTESIAN_POINT ( 'NONE',  ( -9.350000000000008527, 12.50000000000000000, -6.148780366869520897 ) ) ;
#30455=CARTESIAN_POINT ( 'NONE',  ( -14.59999999999998366, 12.50000000000000000, -0.7579135962115894909 ) ) ;
#30456=DIRECTION ( 'NONE',  ( 0.000000000000000000, 0.000000000000000000, 1.000000000000000000 ) ) ;
#30457=ORIENTED_EDGE ( 'NONE', *, *, #50107, .F. ) ;
#30458=ORIENTED_EDGE ( 'NONE', *, *, #51941, .F. ) ;
#30459=AXIS2_PLACEMENT_3D ( 'NONE', #103886, #112424, #22768 ) ;
#30460=EDGE_LOOP ( 'NONE', ( #16023, #45980, #111157, #33765 ) ) ;
#30461=ORIENTED_EDGE ( 'NONE', *, *, #112660, .F. ) ;
#30462=FACE_OUTER_BOUND ( 'NONE', #21897, .T. ) ;
#30463=DIRECTION ( 'NONE',  ( 0.000000000000000000, 1.000000000000000000, 0.000000000000000000 ) ) ;
#30464=EDGE_LOOP ( 'NONE', ( #559, #123221 ) ) ;
#30465=FACE_BOUND ( 'NONE', #52281, .T. ) ;
#30466=CIRCLE ( 'NONE', #65935, 0.06509327318403745899 ) ;
#30467=DIRECTION ( 'NONE',  ( 0.000000000000000000, -0.000000000000000000, 1.000000000000000000 ) ) ;
#30468=CARTESIAN_POINT ( 'NONE',  ( 5.849999999999931255, 2.500000000000000000, 2.757883832488649656 ) ) ;
#30469=VECTOR ( 'NONE', #52661, 1000.000000000000000 ) ;
#30470=DIRECTION ( 'NONE',  ( 0.000000000000000000, 1.000000000000000000, 0.000000000000000000 ) ) ;
#30471=CIRCLE ( 'NONE', #49248, 0.1000000000000002554 ) ;
#30472=DIRECTION ( 'NONE',  ( 0.000000000000000000, 0.000000000000000000, 1.000000000000000000 ) ) ;
#30473=DIRECTION ( 'NONE',  ( 0.000000000000000000, 1.000000000000000000, 0.000000000000000000 ) ) ;
#30474=DIRECTION ( 'NONE',  ( -4.274815082592931898E-19, -0.9999939076577903929, -0.003490651415223739937 ) ) ;
#30475=CARTESIAN_POINT ( 'NONE',  ( -9.350000000000006750, 2.500000000000000000, -1.818653347947325916 ) ) ;
#30476=DIRECTION ( 'NONE',  ( -0.000000000000000000, -1.000000000000000000, -0.000000000000000000 ) ) ;
#30477=VERTEX_POINT ( 'NONE', #35526 ) ;
#30478=CONICAL_SURFACE ( 'NONE', #24199, 0.09999999999999982514, 0.003490658503988666988 ) ;
#30479=ORIENTED_EDGE ( 'NONE', *, *, #110647, .F. ) ;
#30480=EDGE_CURVE ( 'NONE', #70719, #62448, #75424, .T. ) ;
#30481=ORIENTED_EDGE ( 'NONE', *, *, #28178, .T. ) ;
#30482=ORIENTED_EDGE ( 'NONE', *, *, #35063, .T. ) ;
#30483=ORIENTED_EDGE ( 'NONE', *, *, #120664, .F. ) ;
#30484=EDGE_LOOP ( 'NONE', ( #15835, #85447 ) ) ;
#30485=CONICAL_SURFACE ( 'NONE', #63911, 0.1000000000000002554, 0.003490658503988666988 ) ;
#30486=LINE ( 'NONE', #112894, #19149 ) ;
#30487=CARTESIAN_POINT ( 'NONE',  ( 7.299999999999924327, 12.50000000000000000, 0.3464101615137735735 ) ) ;
#30488=EDGE_LOOP ( 'NONE', ( #44519, #25932, #66090, #75890 ) ) ;
#30489=CARTESIAN_POINT ( 'NONE',  ( 15.39999999999989022, 12.50000000000000000, -2.385244779468109755E-15 ) ) ;
#30490=CIRCLE ( 'NONE', #45147, 0.06509327318403745899 ) ;
#30491=VECTOR ( 'NONE', #40118, 1000.000000000000000 ) ;
#30492=EDGE_CURVE ( 'NONE', #25624, #120397, #95134, .T. ) ;
#30493=AXIS2_PLACEMENT_3D ( 'NONE', #49340, #19863, #31615 ) ;
#30494=CARTESIAN_POINT ( 'NONE',  ( 20.37757664703730853, 0.6627606010239018852, 4.188167776336779724 ) ) ;
#30496=CARTESIAN_POINT ( 'NONE',  ( -6.900000000000019007, 2.500000000000000000, -0.3464101615137783474 ) ) ;
#30497=DIRECTION ( 'NONE',  ( 0.000000000000000000, 1.000000000000000000, 0.000000000000000000 ) ) ;
#30498=VECTOR ( 'NONE', #2653, 1000.000000000000000 ) ;
#30499=EDGE_CURVE ( 'NONE', #51256, #72103, #6036, .T. ) ;
#30500=ADVANCED_FACE ( 'NONE', ( #31817 ), #107656, .T. ) ;
#30501=VERTEX_POINT ( 'NONE', #81559 ) ;
#30502=DIRECTION ( 'NONE',  ( -0.000000000000000000, 1.000000000000000000, -0.000000000000000000 ) ) ;
#30503=EDGE_LOOP ( 'NONE', ( #16636, #70052 ) ) ;
#30504=ORIENTED_EDGE ( 'NONE', *, *, #71243, .T. ) ;
#30505=DIRECTION ( 'NONE',  ( -4.274815082592931898E-19, -0.9999939076577903929, -0.003490651415223739937 ) ) ;
#30506=EDGE_CURVE ( 'NONE', #121812, #121834, #59662, .T. ) ;
#30507=CARTESIAN_POINT ( 'NONE',  ( 11.04999999999991189, 12.50000000000000000, -2.576566944158915184 ) ) ;
#30508=FACE_OUTER_BOUND ( 'NONE', #122318, .T. ) ;
#30509=EDGE_CURVE ( 'NONE', #82230, #115626, #94419, .T. ) ;
#30510=CONICAL_SURFACE ( 'NONE', #24227, 0.1000000000000002554, 0.003490658503988666988 ) ;
#30511=ORIENTED_EDGE ( 'NONE', *, *, #37959, .T. ) ;
#30512=ORIENTED_EDGE ( 'NONE', *, *, #96139, .T. ) ;
#30513=FACE_OUTER_BOUND ( 'NONE', #116532, .T. ) ;
#30514=CARTESIAN_POINT ( 'NONE',  ( -10.45000000000000107, 2.500000000000000000, 6.495190528383297135 ) ) ;
#30515=CARTESIAN_POINT ( 'NONE',  ( 0.5999999999999560130, 2.500000000000000000, -3.883716857408426648 ) ) ;
#30516=PLANE ( 'NONE',  #110908 ) ;
#30517=EDGE_LOOP ( 'NONE', ( #66036, #43 ) ) ;
#30518=DIRECTION ( 'NONE',  ( 0.000000000000000000, 0.000000000000000000, 1.000000000000000000 ) ) ;
#30519=CONICAL_SURFACE ( 'NONE', #99462, 0.1000000000000002554, 0.003490658503988666988 ) ;
#30520=AXIS2_PLACEMENT_3D ( 'NONE', #78088, #109480, #80014 ) ;
#30521=ORIENTED_EDGE ( 'NONE', *, *, #116070, .T. ) ;
#30522=FACE_OUTER_BOUND ( 'NONE', #1583, .T. ) ;
#30523=CIRCLE ( 'NONE', #124588, 0.09999999999999982514 ) ;
#30524=VERTEX_POINT ( 'NONE', #16496 ) ;
#30525=CIRCLE ( 'NONE', #28454, 0.06509327318403745899 ) ;
#30526=CARTESIAN_POINT ( 'NONE',  ( -10.20000000000000639, 12.50000000000000000, -3.983716857408421852 ) ) ;
#30527=DIRECTION ( 'NONE',  ( 0.000000000000000000, 0.000000000000000000, 1.000000000000000000 ) ) ;
#30529=DIRECTION ( 'NONE',  ( -0.000000000000000000, -1.000000000000000000, -0.000000000000000000 ) ) ;
#30530=VERTEX_POINT ( 'NONE', #115333 ) ;
#30531=CIRCLE ( 'NONE', #11626, 0.06509327318403745899 ) ;
#30532=FACE_OUTER_BOUND ( 'NONE', #32126, .T. ) ;
#30533=AXIS2_PLACEMENT_3D ( 'NONE', #82630, #102885, #103556 ) ;
#30534=CARTESIAN_POINT ( 'NONE',  ( -14.99999999999998401, 12.50000000000000000, 0.6928203230275518099 ) ) ;
#30535=EDGE_LOOP ( 'NONE', ( #98104, #47737 ) ) ;
#30536=ORIENTED_EDGE ( 'NONE', *, *, #98939, .T. ) ;
#30537=ORIENTED_EDGE ( 'NONE', *, *, #3513, .T. ) ;
#30538=DIRECTION ( 'NONE',  ( 0.000000000000000000, 0.000000000000000000, 1.000000000000000000 ) ) ;
#30539=DIRECTION ( 'NONE',  ( 0.000000000000000000, 1.000000000000000000, 0.000000000000000000 ) ) ;
#30540=DIRECTION ( 'NONE',  ( 0.000000000000000000, 0.000000000000000000, -1.000000000000000000 ) ) ;
#30542=DIRECTION ( 'NONE',  ( 0.000000000000000000, 0.000000000000000000, 1.000000000000000000 ) ) ;
#30543=CARTESIAN_POINT ( 'NONE',  ( -8.350000000000013856, 12.50000000000000000, -5.802370205355744659 ) ) ;
#30544=CIRCLE ( 'NONE', #90871, 0.1000000000000002554 ) ;
#30545=AXIS2_PLACEMENT_3D ( 'NONE', #2761, #81338, #13215 ) ;
#30546=DIRECTION ( 'NONE',  ( 0.000000000000000000, -0.000000000000000000, 1.000000000000000000 ) ) ;
#30547=CARTESIAN_POINT ( 'NONE',  ( -6.250000000000019540, 12.50000000000000000, -2.792790559304616504 ) ) ;
#30548=CARTESIAN_POINT ( 'NONE',  ( 6.049999999999934097, 2.500000000000000000, -6.248780366869526759 ) ) ;
#30549=EDGE_CURVE ( 'NONE', #114181, #21644, #25683, .T. ) ;
#30550=EDGE_CURVE ( 'NONE', #118813, #79023, #51236, .T. ) ;
#30551=EDGE_CURVE ( 'NONE', #91650, #60027, #124383, .T. ) ;
#30552=ADVANCED_FACE ( 'NONE', ( #64959 ), #82621, .T. ) ;
#30553=ORIENTED_EDGE ( 'NONE', *, *, #18952, .F. ) ;
#30554=EDGE_CURVE ( 'NONE', #34203, #80417, #88868, .T. ) ;
#30555=DIRECTION ( 'NONE',  ( 0.000000000000000000, 0.000000000000000000, 1.000000000000000000 ) ) ;
#30556=DIRECTION ( 'NONE',  ( 0.000000000000000000, 1.000000000000000000, 0.000000000000000000 ) ) ;
#30557=CARTESIAN_POINT ( 'NONE',  ( -4.350000000000023626, 12.50000000000000000, -2.446380397790840266 ) ) ;
#30558=DIRECTION ( 'NONE',  ( -0.000000000000000000, 1.000000000000000000, -0.000000000000000000 ) ) ;
#30559=ORIENTED_EDGE ( 'NONE', *, *, #113168, .T. ) ;
#30560=EDGE_CURVE ( 'NONE', #43603, #53182, #1040, .T. ) ;
#30561=DIRECTION ( 'NONE',  ( 0.000000000000000000, 0.000000000000000000, 1.000000000000000000 ) ) ;
#30562=EDGE_CURVE ( 'NONE', #46924, #96072, #53375, .T. ) ;
#30563=AXIS2_PLACEMENT_3D ( 'NONE', #60431, #72813, #11941 ) ;
#30564=AXIS2_PLACEMENT_3D ( 'NONE', #45834, #16338, #96197 ) ;
#30565=CARTESIAN_POINT ( 'NONE',  ( -6.505213034913026604E-15, 2.500000000000000000, 4.330127018922196314 ) ) ;
#30566=CARTESIAN_POINT ( 'NONE',  ( -3.300000000000027800, 2.500000000000000000, 0.09999999999999772959 ) ) ;
#30567=VERTEX_POINT ( 'NONE', #41658 ) ;
#30568=ORIENTED_EDGE ( 'NONE', *, *, #80383, .T. ) ;
#30569=CONICAL_SURFACE ( 'NONE', #24286, 0.09999999999999982514, 0.003490658503988666988 ) ;
#30570=FACE_OUTER_BOUND ( 'NONE', #36137, .T. ) ;
#30571=ORIENTED_EDGE ( 'NONE', *, *, #35687, .T. ) ;
#30572=VERTEX_POINT ( 'NONE', #85881 ) ;
#30573=DIRECTION ( 'NONE',  ( 0.000000000000000000, -0.000000000000000000, 1.000000000000000000 ) ) ;
#30574=CARTESIAN_POINT ( 'NONE',  ( 18.87984495337804347, 0.5408627091912223683, -4.542689527608963829 ) ) ;
#30575=FACE_OUTER_BOUND ( 'NONE', #80956, .T. ) ;
#30576=CIRCLE ( 'NONE', #39000, 0.1000000000000002554 ) ;
#30577=DIRECTION ( 'NONE',  ( 0.000000000000000000, 0.000000000000000000, 1.000000000000000000 ) ) ;
#30578=ORIENTED_EDGE ( 'NONE', *, *, #46470, .F. ) ;
#30579=CIRCLE ( 'NONE', #126708, 0.06509327318403745899 ) ;
#30580=PLANE ( 'NONE',  #23138 ) ;
#30581=VERTEX_POINT ( 'NONE', #125807 ) ;
#30582=CARTESIAN_POINT ( 'NONE',  ( 8.349999999999923261, 2.500000000000000000, -7.088010851410853519 ) ) ;
#30583=DIRECTION ( 'NONE',  ( -0.000000000000000000, -1.000000000000000000, -0.000000000000000000 ) ) ;
#30584=EDGE_CURVE ( 'NONE', #36319, #41518, #64326, .T. ) ;
#30585=CARTESIAN_POINT ( 'NONE',  ( 17.10613367507967553, -2.036230694789212592, 5.376205058613408028 ) ) ;
#30586=ORIENTED_EDGE ( 'NONE', *, *, #17167, .T. ) ;
#30587=ORIENTED_EDGE ( 'NONE', *, *, #84611, .T. ) ;
#30588=ORIENTED_EDGE ( 'NONE', *, *, #120786, .T. ) ;
#30589=ORIENTED_EDGE ( 'NONE', *, *, #84984, .T. ) ;
#30590=EDGE_LOOP ( 'NONE', ( #92254, #89348 ) ) ;
#30591=LINE ( 'NONE', #61969, #62867 ) ;
#30592=DIRECTION ( 'NONE',  ( -4.274815082592931898E-19, -0.9999939076577903929, -0.003490651415223739937 ) ) ;
#30593=DIRECTION ( 'NONE',  ( -0.000000000000000000, -1.000000000000000000, -0.000000000000000000 ) ) ;
#30594=FACE_BOUND ( 'NONE', #9947, .T. ) ;
#30595=FACE_OUTER_BOUND ( 'NONE', #119200, .T. ) ;
#30596=CONICAL_SURFACE ( 'NONE', #26469, 0.1000000000000000472, 0.003490658503988666988 ) ;
#30597=FACE_OUTER_BOUND ( 'NONE', #120146, .T. ) ;
#30598=FACE_OUTER_BOUND ( 'NONE', #44238, .T. ) ;
#30599=DIRECTION ( 'NONE',  ( -0.000000000000000000, 1.000000000000000000, -0.000000000000000000 ) ) ;
#30600=EDGE_CURVE ( 'NONE', #89491, #56415, #85257, .T. ) ;
#30601=CIRCLE ( 'NONE', #118592, 0.1000000000000002554 ) ;
#30602=LINE ( 'NONE', #89502, #25498 ) ;
#30603=AXIS2_PLACEMENT_3D ( 'NONE', #45763, #35930, #22903 ) ;
#30604=DIRECTION ( 'NONE',  ( 0.000000000000000000, 0.000000000000000000, 1.000000000000000000 ) ) ;
#30605=DIRECTION ( 'NONE',  ( 0.000000000000000000, 0.000000000000000000, 1.000000000000000000 ) ) ;
#30606=AXIS2_PLACEMENT_3D ( 'NONE', #109144, #119616, #99996 ) ;
#30607=CIRCLE ( 'NONE', #120472, 0.06509327318403745899 ) ;
#30608=CARTESIAN_POINT ( 'NONE',  ( 11.89999999999990798, 12.50000000000000000, -4.048810130592463530 ) ) ;
#30609=CIRCLE ( 'NONE', #120475, 0.1000000000000002554 ) ;
#30610=ORIENTED_EDGE ( 'NONE', *, *, #118435, .F. ) ;
#30611=VERTEX_POINT ( 'NONE', #76726 ) ;
#30612=ORIENTED_EDGE ( 'NONE', *, *, #58291, .T. ) ;
#30613=ORIENTED_EDGE ( 'NONE', *, *, #27340, .T. ) ;
#30614=CARTESIAN_POINT ( 'NONE',  ( -0.4000000000000401013, 12.50000000000000000, -3.637306695894650055 ) ) ;
#30615=DIRECTION ( 'NONE',  ( 0.000000000000000000, 0.000000000000000000, -1.000000000000000000 ) ) ;
#30616=FACE_BOUND ( 'NONE', #99031, .T. ) ;
#30617=AXIS2_PLACEMENT_3D ( 'NONE', #59418, #109784, #20113 ) ;
#30618=DIRECTION ( 'NONE',  ( 0.000000000000000000, 0.000000000000000000, 1.000000000000000000 ) ) ;
#30619=CONICAL_SURFACE ( 'NONE', #82850, 0.1000000000000002554, 0.003490658503988666988 ) ;
#30620=CONICAL_SURFACE ( 'NONE', #103767, 0.1000000000000000472, 0.003490658503988666988 ) ;
#30621=EDGE_LOOP ( 'NONE', ( #7468, #65999, #21886, #73625 ) ) ;
#30622=FACE_OUTER_BOUND ( 'NONE', #18504, .T. ) ;
#30623=DIRECTION ( 'NONE',  ( 0.000000000000000000, 1.000000000000000000, 0.000000000000000000 ) ) ;
#30624=DIRECTION ( 'NONE',  ( 0.000000000000000000, 0.000000000000000000, -1.000000000000000000 ) ) ;
#30625=DIRECTION ( 'NONE',  ( 0.000000000000000000, 0.000000000000000000, -1.000000000000000000 ) ) ;
#30626=ORIENTED_EDGE ( 'NONE', *, *, #17973, .T. ) ;
#30627=CARTESIAN_POINT ( 'NONE',  ( -12.49999999999999289, 2.500000000000000000, -5.122947341949751987 ) ) ;
#30628=ORIENTED_EDGE ( 'NONE', *, *, #44258, .F. ) ;
#30629=EDGE_LOOP ( 'NONE', ( #116806, #35857 ) ) ;
#30630=CARTESIAN_POINT ( 'NONE',  ( 12.89999999999990088, 2.500000000000000000, 4.330127018922196314 ) ) ;
#30631=CARTESIAN_POINT ( 'NONE',  ( -1.250000000000001110, 12.50000000000000000, -2.099970236277064473 ) ) ;
#30632=EDGE_LOOP ( 'NONE', ( #30683, #45576, #115214, #81854 ) ) ;
#30633=DIRECTION ( 'NONE',  ( 0.000000000000000000, 1.000000000000000000, 0.000000000000000000 ) ) ;
#30634=EDGE_CURVE ( 'NONE', #46379, #67379, #32471, .T. ) ;
#30635=DIRECTION ( 'NONE',  ( -0.000000000000000000, -1.000000000000000000, -0.000000000000000000 ) ) ;
#30636=FACE_OUTER_BOUND ( 'NONE', #69536, .T. ) ;
#30637=DIRECTION ( 'NONE',  ( 0.000000000000000000, 0.000000000000000000, 1.000000000000000000 ) ) ;
#30638=VERTEX_POINT ( 'NONE', #78010 ) ;
#30639=EDGE_CURVE ( 'NONE', #7770, #120491, #57744, .T. ) ;
#30640=DIRECTION ( 'NONE',  ( -0.000000000000000000, -1.000000000000000000, -0.000000000000000000 ) ) ;
#30641=EDGE_CURVE ( 'NONE', #41537, #29412, #99343, .T. ) ;
#30643=CARTESIAN_POINT ( 'NONE',  ( -1.900000000000034550, 2.500000000000000000, 4.676537180435972552 ) ) ;
#30644=VERTEX_POINT ( 'NONE', #86540 ) ;
#30645=VECTOR ( 'NONE', #98140, 1000.000000000000000 ) ;
#30646=FACE_OUTER_BOUND ( 'NONE', #64338, .T. ) ;
#30647=ORIENTED_EDGE ( 'NONE', *, *, #32747, .T. ) ;
#30648=DIRECTION ( 'NONE',  ( 0.000000000000000000, 0.000000000000000000, -1.000000000000000000 ) ) ;
#30649=CARTESIAN_POINT ( 'NONE',  ( -0.6000000000000323963, 2.500000000000000000, 0.4464101615137759382 ) ) ;
#30650=EDGE_CURVE ( 'NONE', #109098, #112569, #89123, .T. ) ;
#30651=ADVANCED_FACE ( 'NONE', ( #26992 ), #19923, .T. ) ;
#30652=DIRECTION ( 'NONE',  ( -0.000000000000000000, -1.000000000000000000, -0.000000000000000000 ) ) ;
#30653=EDGE_CURVE ( 'NONE', #79005, #95802, #44966, .T. ) ;
#30654=DIRECTION ( 'NONE',  ( -4.274815082592931898E-19, -0.9999939076577903929, -0.003490651415223739937 ) ) ;
#30655=EDGE_CURVE ( 'NONE', #5036, #115994, #93085, .T. ) ;
#30656=EDGE_CURVE ( 'NONE', #119339, #111925, #19069, .T. ) ;
#30657=DIRECTION ( 'NONE',  ( 0.000000000000000000, -0.000000000000000000, 1.000000000000000000 ) ) ;
#30658=VERTEX_POINT ( 'NONE', #29557 ) ;
#30659=CIRCLE ( 'NONE', #68280, 0.06509327318403745899 ) ;
#30660=AXIS2_PLACEMENT_3D ( 'NONE', #56010, #78751, #146 ) ;
#30661=ORIENTED_EDGE ( 'NONE', *, *, #97923, .F. ) ;
#30662=ORIENTED_EDGE ( 'NONE', *, *, #1546, .T. ) ;
#30663=CARTESIAN_POINT ( 'NONE',  ( -2.700000000000030820, 2.500000000000000000, 0.4464101615137735513 ) ) ;
#30664=DIRECTION ( 'NONE',  ( -0.000000000000000000, 1.000000000000000000, -0.000000000000000000 ) ) ;
#30666=EDGE_LOOP ( 'NONE', ( #96628, #34839, #19452, #126456 ) ) ;
#30667=ORIENTED_EDGE ( 'NONE', *, *, #78717, .F. ) ;
#30668=VERTEX_POINT ( 'NONE', #36814 ) ;
#30669=ADVANCED_FACE ( 'NONE', ( #27603 ), #5235, .T. ) ;
#30670=CARTESIAN_POINT ( 'NONE',  ( -6.850000000000017408, 12.50000000000000000, -2.446380397790840266 ) ) ;
#30671=CIRCLE ( 'NONE', #122676, 0.06509327318403745899 ) ;
#30672=AXIS2_PLACEMENT_3D ( 'NONE', #111366, #1425, #92382 ) ;
#30673=ORIENTED_EDGE ( 'NONE', *, *, #87344, .T. ) ;
#30674=CARTESIAN_POINT ( 'NONE',  ( -7.700000000000016165, 2.500000000000000000, -3.983716857408426293 ) ) ;
#30675=AXIS2_PLACEMENT_3D ( 'NONE', #126282, #37891, #97459 ) ;
#30676=DIRECTION ( 'NONE',  ( 0.000000000000000000, 0.000000000000000000, 1.000000000000000000 ) ) ;
#30677=DIRECTION ( 'NONE',  ( -0.000000000000000000, 1.000000000000000000, -0.000000000000000000 ) ) ;
#30678=CARTESIAN_POINT ( 'NONE',  ( -3.750000000000025757, 2.500000000000000000, -2.857883832488653741 ) ) ;
#30679=LINE ( 'NONE', #10996, #57637 ) ;
#30680=DIRECTION ( 'NONE',  ( -0.000000000000000000, 1.000000000000000000, -0.000000000000000000 ) ) ;
#30681=DIRECTION ( 'NONE',  ( -0.000000000000000000, -1.000000000000000000, -0.000000000000000000 ) ) ;
#30682=VERTEX_POINT ( 'NONE', #119226 ) ;
#30683=ORIENTED_EDGE ( 'NONE', *, *, #9016, .T. ) ;
#30684=CARTESIAN_POINT ( 'NONE',  ( 0.1999999999999562961, 12.50000000000000000, 4.611443907251934426 ) ) ;
#30685=CARTESIAN_POINT ( 'NONE',  ( 4.399999999999940847, 12.50000000000000000, -4.676537180435977881 ) ) ;
#30687=ORIENTED_EDGE ( 'NONE', *, *, #103374, .F. ) ;
#30689=CARTESIAN_POINT ( 'NONE',  ( 14.39999999999989555, 2.500000000000000000, 0.3464101615137736845 ) ) ;
#30690=VECTOR ( 'NONE', #125443, 1000.000000000000000 ) ;
#30691=FACE_OUTER_BOUND ( 'NONE', #82948, .T. ) ;
#30692=DIRECTION ( 'NONE',  ( 0.000000000000000000, 1.000000000000000000, 0.000000000000000000 ) ) ;
#30693=CIRCLE ( 'NONE', #26471, 0.1000000000000002554 ) ;
#30694=CARTESIAN_POINT ( 'NONE',  ( -1.250000000000037526, 12.50000000000000000, -1.537336459617587581 ) ) ;
#30695=FACE_OUTER_BOUND ( 'NONE', #43984, .T. ) ;
#30696=AXIS2_PLACEMENT_3D ( 'NONE', #111543, #90605, #946 ) ;
#30697=CARTESIAN_POINT ( 'NONE',  ( 7.099999999999927702, 12.50000000000000000, -3.572213422710612374 ) ) ;
#30698=DIRECTION ( 'NONE',  ( 0.000000000000000000, 1.000000000000000000, 0.000000000000000000 ) ) ;
#30699=ADVANCED_FACE ( 'NONE', ( #107476 ), #97007, .T. ) ;
#30700=AXIS2_PLACEMENT_3D ( 'NONE', #38349, #128003, #66494 ) ;
#30701=ADVANCED_FACE ( 'NONE', ( #47278 ), #7375, .T. ) ;
#30702=AXIS2_PLACEMENT_3D ( 'NONE', #58144, #88202, #18841 ) ;
#30703=LINE ( 'NONE', #11677, #83509 ) ;
#30704=ORIENTED_EDGE ( 'NONE', *, *, #50894, .F. ) ;
#30705=ORIENTED_EDGE ( 'NONE', *, *, #123478, .F. ) ;
#30706=AXIS2_PLACEMENT_3D ( 'NONE', #91722, #91074, #89786 ) ;
#30707=ADVANCED_FACE ( 'NONE', ( #98286 ), #47199, .T. ) ;
#30708=EDGE_LOOP ( 'NONE', ( #38069, #108944 ) ) ;
#30709=ORIENTED_EDGE ( 'NONE', *, *, #86204, .F. ) ;
#30710=CIRCLE ( 'NONE', #7683, 0.09999999999999999167 ) ;
#30711=EDGE_CURVE ( 'NONE', #40465, #25579, #8602, .T. ) ;
#30712=EDGE_LOOP ( 'NONE', ( #129094, #8180 ) ) ;
#30713=FACE_OUTER_BOUND ( 'NONE', #111699, .T. ) ;
#30714=DIRECTION ( 'NONE',  ( 0.000000000000000000, 1.000000000000000000, 0.000000000000000000 ) ) ;
#30715=CIRCLE ( 'NONE', #41088, 0.06509327318403745899 ) ;
#30717=ORIENTED_EDGE ( 'NONE', *, *, #52066, .F. ) ;
#30718=EDGE_CURVE ( 'NONE', #62072, #11437, #128431, .T. ) ;
#30719=FACE_OUTER_BOUND ( 'NONE', #64753, .T. ) ;
#30720=DIRECTION ( 'NONE',  ( -0.000000000000000000, -1.000000000000000000, -0.000000000000000000 ) ) ;
#30721=CIRCLE ( 'NONE', #26498, 0.1000000000000000056 ) ;
#30722=VECTOR ( 'NONE', #93571, 1000.000000000000000 ) ;
#30723=EDGE_CURVE ( 'NONE', #67433, #52089, #28274, .T. ) ;
#30724=DIRECTION ( 'NONE',  ( 0.000000000000000000, -0.9999939076577903929, 0.003490651415223739937 ) ) ;
#30725=CARTESIAN_POINT ( 'NONE',  ( -8.350000000000013856, 2.500000000000000000, 2.265063509461097357 ) ) ;
#30726=EDGE_LOOP ( 'NONE', ( #39797, #104361 ) ) ;
#30727=CARTESIAN_POINT ( 'NONE',  ( 5.199999999999931788, 2.500000000000000000, 4.676537180435972552 ) ) ;
#30728=ADVANCED_FACE ( 'NONE', ( #69469 ), #72253, .T. ) ;
#30729=CARTESIAN_POINT ( 'NONE',  ( -3.550000000000027800, 2.500000000000000000, 6.248780366869520542 ) ) ;
#30730=EDGE_LOOP ( 'NONE', ( #14069, #28254 ) ) ;
#30731=ORIENTED_EDGE ( 'NONE', *, *, #40337, .T. ) ;
#30732=EDGE_LOOP ( 'NONE', ( #45937, #111915, #128542, #5804 ) ) ;
#30733=ORIENTED_EDGE ( 'NONE', *, *, #104925, .T. ) ;
#30734=CARTESIAN_POINT ( 'NONE',  ( -10.65000000000000391, 2.500000000000000000, -6.148780366869522673 ) ) ;
#30735=CIRCLE ( 'NONE', #13966, 0.06509327318403741736 ) ;
#30736=DIRECTION ( 'NONE',  ( -4.274815082592931898E-19, -0.9999939076577903929, -0.003490651415223739937 ) ) ;
#30737=CARTESIAN_POINT ( 'NONE',  ( 7.499999999999960032, 2.500000000000000000, -2.276824562219559311E-15 ) ) ;
#30738=CARTESIAN_POINT ( 'NONE',  ( -8.350000000000013856, 2.500000000000000000, -2.065063509461102065 ) ) ;
#30739=ORIENTED_EDGE ( 'NONE', *, *, #27456, .T. ) ;
#30740=CARTESIAN_POINT ( 'NONE',  ( -1.700000000000034817, 12.50000000000000000, 0.06509327318403504425 ) ) ;
#30741=CARTESIAN_POINT ( 'NONE',  ( 18.29531403502781828, -0.5011766475904796403, -4.780851392375756070 ) ) ;
#30742=LINE ( 'NONE', #70639, #94378 ) ;
#30743=CARTESIAN_POINT ( 'NONE',  ( -11.44999999999999751, 2.500000000000000000, 1.918653347947321564 ) ) ;
#30744=ADVANCED_FACE ( 'NONE', ( #100238 ), #55516, .T. ) ;
#30745=VERTEX_POINT ( 'NONE', #80601 ) ;
#30747=CARTESIAN_POINT ( 'NONE',  ( 6.049999999999935874, 12.50000000000000000, -6.841600689897077814 ) ) ;
#30748=CONICAL_SURFACE ( 'NONE', #106032, 0.1000000000000000472, 0.003490658503988666988 ) ;
#30749=ORIENTED_EDGE ( 'NONE', *, *, #92853, .T. ) ;
#30750=VERTEX_POINT ( 'NONE', #102169 ) ;
#30751=CARTESIAN_POINT ( 'NONE',  ( 6.699999999999930012, 12.50000000000000000, 4.265033745738159077 ) ) ;
#30752=DIRECTION ( 'NONE',  ( 0.000000000000000000, 0.000000000000000000, -1.000000000000000000 ) ) ;
#30753=FACE_BOUND ( 'NONE', #7270, .T. ) ;
#30754=CARTESIAN_POINT ( 'NONE',  ( -10.80000000000000071, 2.500000000000000000, 4.230127018922196669 ) ) ;
#30755=DIRECTION ( 'NONE',  ( 0.000000000000000000, 0.000000000000000000, -1.000000000000000000 ) ) ;
#30756=CIRCLE ( 'NONE', #93428, 0.06509327318403745899 ) ;
#30757=CARTESIAN_POINT ( 'NONE',  ( 13.29999999999989946, 2.500000000000000000, -0.1000000000000023925 ) ) ;
#30758=EDGE_CURVE ( 'NONE', #110183, #99983, #100862, .T. ) ;
#30759=DIRECTION ( 'NONE',  ( -0.000000000000000000, -1.000000000000000000, -0.000000000000000000 ) ) ;
#30760=DIRECTION ( 'NONE',  ( 0.000000000000000000, 1.000000000000000000, 0.000000000000000000 ) ) ;
#30761=CARTESIAN_POINT ( 'NONE',  ( -6.450000000000017941, 2.500000000000000000, -2.511473670974877948 ) ) ;
#30762=ORIENTED_EDGE ( 'NONE', *, *, #30509, .F. ) ;
#30763=AXIS2_PLACEMENT_3D ( 'NONE', #90740, #12161, #111677 ) ;
#30764=CONICAL_SURFACE ( 'NONE', #103903, 0.09999999999999982514, 0.003490658503988666988 ) ;
#30765=CARTESIAN_POINT ( 'NONE',  ( 5.649999999999932854, 2.500000000000000000, 1.718653347947321386 ) ) ;
#30766=VECTOR ( 'NONE', #22576, 1000.000000000000000 ) ;
#30767=DIRECTION ( 'NONE',  ( -4.274815082592931898E-19, -0.9999939076577903929, -0.003490651415223739937 ) ) ;
#30768=ORIENTED_EDGE ( 'NONE', *, *, #9231, .F. ) ;
#30769=ORIENTED_EDGE ( 'NONE', *, *, #28645, .F. ) ;
#30770=CARTESIAN_POINT ( 'NONE',  ( -4.150000000000025224, 2.500000000000000000, -1.472243186433550122 ) ) ;
#30771=EDGE_CURVE ( 'NONE', #37867, #81193, #126628, .T. ) ;
#30772=FACE_OUTER_BOUND ( 'NONE', #76910, .T. ) ;
#30773=FACE_BOUND ( 'NONE', #7015, .T. ) ;
#30774=DIRECTION ( 'NONE',  ( 0.000000000000000000, 0.000000000000000000, 1.000000000000000000 ) ) ;
#30775=DIRECTION ( 'NONE',  ( 0.000000000000000000, 1.000000000000000000, 0.000000000000000000 ) ) ;
#30776=EDGE_LOOP ( 'NONE', ( #26143, #26240, #4321, #117650 ) ) ;
#30777=DIRECTION ( 'NONE',  ( 0.000000000000000000, 1.000000000000000000, 0.000000000000000000 ) ) ;
#30779=CIRCLE ( 'NONE', #93457, 0.09999999999999999167 ) ;
#30780=ORIENTED_EDGE ( 'NONE', *, *, #108452, .T. ) ;
#30781=DIRECTION ( 'NONE',  ( 0.000000000000000000, -0.000000000000000000, 1.000000000000000000 ) ) ;
#30782=AXIS2_PLACEMENT_3D ( 'NONE', #125742, #24353, #95665 ) ;
#30783=LINE ( 'NONE', #70686, #7326 ) ;
#30784=AXIS2_PLACEMENT_3D ( 'NONE', #86584, #95133, #96397 ) ;
#30785=LINE ( 'NONE', #61530, #69488 ) ;
#30786=FACE_OUTER_BOUND ( 'NONE', #18603, .T. ) ;
#30787=AXIS2_PLACEMENT_3D ( 'NONE', #48816, #89998, #58635 ) ;
#30788=AXIS2_PLACEMENT_3D ( 'NONE', #126722, #36424, #75666 ) ;
#30789=VERTEX_POINT ( 'NONE', #91703 ) ;
#30790=EDGE_CURVE ( 'NONE', #53425, #77768, #111961, .T. ) ;
#30791=DIRECTION ( 'NONE',  ( -0.000000000000000000, 1.000000000000000000, -0.000000000000000000 ) ) ;
#30792=DIRECTION ( 'NONE',  ( 0.000000000000000000, -0.000000000000000000, 1.000000000000000000 ) ) ;
#30793=DIRECTION ( 'NONE',  ( 0.000000000000000000, 0.000000000000000000, 1.000000000000000000 ) ) ;
#30794=ORIENTED_EDGE ( 'NONE', *, *, #122112, .T. ) ;
#30795=EDGE_LOOP ( 'NONE', ( #111399, #16255, #125117, #78612 ) ) ;
#30796=AXIS2_PLACEMENT_3D ( 'NONE', #128205, #78476, #1812 ) ;
#30797=DIRECTION ( 'NONE',  ( 0.000000000000000000, -0.000000000000000000, 1.000000000000000000 ) ) ;
#30798=ADVANCED_FACE ( 'NONE', ( #70139 ), #12488, .T. ) ;
#30799=ORIENTED_EDGE ( 'NONE', *, *, #20561, .T. ) ;
#30800=CARTESIAN_POINT ( 'NONE',  ( 11.04999999999991012, 2.500000000000000000, -1.818653347947326138 ) ) ;
#30801=CARTESIAN_POINT ( 'NONE',  ( 17.50000000000000000, -2.499999999999999556, 1.666666666666671404 ) ) ;
#30802=CONICAL_SURFACE ( 'NONE', #45473, 0.09999999999999982514, 0.003490658503988666988 ) ;
#30803=AXIS2_PLACEMENT_3D ( 'NONE', #24027, #83595, #93407 ) ;
#30804=FACE_OUTER_BOUND ( 'NONE', #72370, .T. ) ;
#30805=ORIENTED_EDGE ( 'NONE', *, *, #59949, .T. ) ;
#30806=CARTESIAN_POINT ( 'NONE',  ( 6.249999999999932498, 2.500000000000000000, -5.802370205355749988 ) ) ;
#30807=DIRECTION ( 'NONE',  ( 0.000000000000000000, -0.000000000000000000, 1.000000000000000000 ) ) ;
#30809=EDGE_CURVE ( 'NONE', #84669, #83875, #32155, .T. ) ;
#30810=EDGE_CURVE ( 'NONE', #109919, #125301, #31494, .T. ) ;
#30811=CARTESIAN_POINT ( 'NONE',  ( 14.14999999999989733, 2.500000000000000000, 1.572243186433545548 ) ) ;
#30812=FACE_OUTER_BOUND ( 'NONE', #44043, .T. ) ;
#30813=ADVANCED_FACE ( 'NONE', ( #40033 ), #88965, .T. ) ;
#30814=ADVANCED_FACE ( 'NONE', ( #60944 ), #11192, .T. ) ;
#30815=CARTESIAN_POINT ( 'NONE',  ( 9.399999999999918643, 12.50000000000000000, 0.3464101615137736845 ) ) ;
#30816=VERTEX_POINT ( 'NONE', #30868 ) ;
#30817=ORIENTED_EDGE ( 'NONE', *, *, #18722, .T. ) ;
#30818=DIRECTION ( 'NONE',  ( 0.000000000000000000, 0.000000000000000000, -1.000000000000000000 ) ) ;
#30819=EDGE_LOOP ( 'NONE', ( #77201, #43194 ) ) ;
#30821=ORIENTED_EDGE ( 'NONE', *, *, #42569, .F. ) ;
#30822=ORIENTED_EDGE ( 'NONE', *, *, #102735, .F. ) ;
#30823=EDGE_LOOP ( 'NONE', ( #79565, #9419 ) ) ;
#30824=AXIS2_PLACEMENT_3D ( 'NONE', #69750, #59965, #109685 ) ;
#30825=ADVANCED_FACE ( 'NONE', ( #72077 ), #101492, .T. ) ;
#30826=CARTESIAN_POINT ( 'NONE',  ( 17.50000000000000000, -2.083333333333331705, -3.999999999999998224 ) ) ;
#30827=ADVANCED_FACE ( 'NONE', ( #101525 ), #7475, .T. ) ;
#30829=ADVANCED_FACE ( 'NONE', ( #41964 ), #40887, .T. ) ;
#30830=DIRECTION ( 'NONE',  ( -0.000000000000000000, -1.000000000000000000, -0.000000000000000000 ) ) ;
#30831=CARTESIAN_POINT ( 'NONE',  ( 14.14999999999989733, 2.500000000000000000, 1.372243186433545370 ) ) ;
#30832=DIRECTION ( 'NONE',  ( 0.000000000000000000, -0.000000000000000000, 1.000000000000000000 ) ) ;
#30833=CARTESIAN_POINT ( 'NONE',  ( -10.40000000000000391, 12.50000000000000000, -3.637306695894645614 ) ) ;
#30834=CARTESIAN_POINT ( 'NONE',  ( -1.450000000000035927, 2.500000000000000000, -1.918653347947326004 ) ) ;
#30835=DIRECTION ( 'NONE',  ( -0.000000000000000000, -1.000000000000000000, -0.000000000000000000 ) ) ;
#30836=CARTESIAN_POINT ( 'NONE',  ( 5.649999999999934630, 12.50000000000000000, -1.818653347947325916 ) ) ;
#30837=CIRCLE ( 'NONE', #114425, 0.1000000000000000056 ) ;
#30838=ORIENTED_EDGE ( 'NONE', *, *, #112833, .T. ) ;
#30839=DIRECTION ( 'NONE',  ( 0.000000000000000000, 1.000000000000000000, 0.000000000000000000 ) ) ;
#30840=ORIENTED_EDGE ( 'NONE', *, *, #86199, .T. ) ;
#30841=VERTEX_POINT ( 'NONE', #36011 ) ;
#30842=DIRECTION ( 'NONE',  ( 0.000000000000000000, 0.000000000000000000, -1.000000000000000000 ) ) ;
#30843=CARTESIAN_POINT ( 'NONE',  ( -2.050000000000032685, 2.500000000000000000, -2.265063509461101798 ) ) ;
#30844=VECTOR ( 'NONE', #56141, 1000.000000000000000 ) ;
#30845=CIRCLE ( 'NONE', #35052, 0.06509327318403745899 ) ;
#30846=VECTOR ( 'NONE', #50595, 1000.000000000000000 ) ;
#30847=DIRECTION ( 'NONE',  ( 0.000000000000000000, 1.000000000000000000, 0.000000000000000000 ) ) ;
#30848=DIRECTION ( 'NONE',  ( 0.000000000000000000, -0.9999939076577903929, 0.003490651415223739937 ) ) ;
#30849=DIRECTION ( 'NONE',  ( 0.000000000000000000, -0.9999939076577903929, 0.003490651415223739937 ) ) ;
#30850=EDGE_LOOP ( 'NONE', ( #54743, #44688 ) ) ;
#30851=CIRCLE ( 'NONE', #107905, 0.09999999999999982514 ) ;
#30852=VERTEX_POINT ( 'NONE', #115174 ) ;
#30853=CARTESIAN_POINT ( 'NONE',  ( 16.56576425165006228, 1.499999999999999556, -6.084390597445811011 ) ) ;
#30854=CONICAL_SURFACE ( 'NONE', #14092, 0.1000000000000002554, 0.003490658503988666988 ) ;
#30855=ORIENTED_EDGE ( 'NONE', *, *, #117507, .T. ) ;
#30857=ORIENTED_EDGE ( 'NONE', *, *, #14444, .T. ) ;
#30858=EDGE_CURVE ( 'NONE', #121003, #126895, #91023, .T. ) ;
#30859=EDGE_LOOP ( 'NONE', ( #34789, #90128, #57327, #60338 ) ) ;
#30860=CARTESIAN_POINT ( 'NONE',  ( 13.09999999999989839, 12.50000000000000000, -0.4115034346978157509 ) ) ;
#30861=DIRECTION ( 'NONE',  ( 0.000000000000000000, 0.000000000000000000, 1.000000000000000000 ) ) ;
#30862=ADVANCED_FACE ( 'NONE', ( #44530 ), #83182, .T. ) ;
#30863=AXIS2_PLACEMENT_3D ( 'NONE', #94516, #116096, #46078 ) ;
#30864=FACE_OUTER_BOUND ( 'NONE', #125415, .T. ) ;
#30865=DIRECTION ( 'NONE',  ( 0.000000000000000000, -0.9999939076577903929, 0.003490651415223739937 ) ) ;
#30866=EDGE_CURVE ( 'NONE', #116963, #43630, #102792, .T. ) ;
#30867=AXIS2_PLACEMENT_3D ( 'NONE', #16610, #76201, #65062 ) ;
#30868=CARTESIAN_POINT ( 'NONE',  ( 3.749999999999942268, 2.500000000000000000, 1.572243186433545548 ) ) ;
#30869=ORIENTED_EDGE ( 'NONE', *, *, #123626, .F. ) ;
#30870=FACE_OUTER_BOUND ( 'NONE', #85760, .T. ) ;
#30871=DIRECTION ( 'NONE',  ( 0.000000000000000000, 0.000000000000000000, 1.000000000000000000 ) ) ;
#30872=CARTESIAN_POINT ( 'NONE',  ( 17.49862860983167323, 2.500000000000000000, -4.081131818001370704 ) ) ;
#30873=CARTESIAN_POINT ( 'NONE',  ( -14.79999999999998295, 2.500000000000000000, -0.4464101615137760493 ) ) ;
#30874=AXIS2_PLACEMENT_3D ( 'NONE', #114491, #24832, #64747 ) ;
#30875=AXIS2_PLACEMENT_3D ( 'NONE', #98006, #118941, #29286 ) ;
#30876=EDGE_CURVE ( 'NONE', #94676, #56167, #83805, .T. ) ;
#30877=DIRECTION ( 'NONE',  ( 0.000000000000000000, 0.000000000000000000, 1.000000000000000000 ) ) ;
#30878=ORIENTED_EDGE ( 'NONE', *, *, #55924, .F. ) ;
#30879=CIRCLE ( 'NONE', #16159, 0.06509327318403745899 ) ;
#30880=VERTEX_POINT ( 'NONE', #113926 ) ;
#30881=CARTESIAN_POINT ( 'NONE',  ( -7.100000000000017408, 2.500000000000000000, 0.6928203230275494784 ) ) ;
#30882=CIRCLE ( 'NONE', #7860, 0.1000000000000002554 ) ;
#30883=EDGE_CURVE ( 'NONE', #118717, #9579, #3285, .T. ) ;
#30884=ORIENTED_EDGE ( 'NONE', *, *, #8713, .F. ) ;
#30885=CIRCLE ( 'NONE', #76844, 0.06509327318403745899 ) ;
#30886=CARTESIAN_POINT ( 'NONE',  ( -14.59999999999998366, 2.500000000000000000, -0.5928203230275519431 ) ) ;
#30887=CARTESIAN_POINT ( 'NONE',  ( -6.650000000000014566, 2.500000000000000000, 2.165063509461097713 ) ) ;
#30888=CIRCLE ( 'NONE', #70574, 0.1000000000000002554 ) ;
#30889=ORIENTED_EDGE ( 'NONE', *, *, #40005, .F. ) ;
#30890=CARTESIAN_POINT ( 'NONE',  ( -3.750000000000025757, 2.500000000000000000, 1.572243186433545548 ) ) ;
#30891=DIRECTION ( 'NONE',  ( -0.000000000000000000, -1.000000000000000000, -0.000000000000000000 ) ) ;
#30892=CONICAL_SURFACE ( 'NONE', #87295, 0.09999999999999982514, 0.003490658503988666988 ) ;
#30893=CARTESIAN_POINT ( 'NONE',  ( 11.84999999999990372, 2.500000000000000000, -6.941600689897078347 ) ) ;
#30894=EDGE_CURVE ( 'NONE', #6638, #74055, #118207, .T. ) ;
#30895=DIRECTION ( 'NONE',  ( 0.000000000000000000, 0.000000000000000000, -1.000000000000000000 ) ) ;
#30896=AXIS2_PLACEMENT_3D ( 'NONE', #30489, #40295, #48172 ) ;
#30897=DIRECTION ( 'NONE',  ( -0.000000000000000000, 1.000000000000000000, -0.000000000000000000 ) ) ;
#30898=ORIENTED_EDGE ( 'NONE', *, *, #31523, .F. ) ;
#30899=CARTESIAN_POINT ( 'NONE',  ( 8.749999999999921840, 2.500000000000000000, -5.702370205355749455 ) ) ;
#30900=CARTESIAN_POINT ( 'NONE',  ( -3.150000000000029665, 2.500000000000000000, 6.741600689897071952 ) ) ;
#30901=DIRECTION ( 'NONE',  ( -4.274815082592931898E-19, -0.9999939076577903929, -0.003490651415223739937 ) ) ;
#30902=DIRECTION ( 'NONE',  ( -4.274815082592931898E-19, -0.9999939076577903929, -0.003490651415223739937 ) ) ;
#30903=ORIENTED_EDGE ( 'NONE', *, *, #89775, .F. ) ;
#30904=ADVANCED_FACE ( 'NONE', ( #64811 ), #51330, .T. ) ;
#30905=ORIENTED_EDGE ( 'NONE', *, *, #56407, .F. ) ;
#30907=CARTESIAN_POINT ( 'NONE',  ( 5.599999999999934808, 12.50000000000000000, -3.983716857408426293 ) ) ;
#30908=CIRCLE ( 'NONE', #37164, 0.06509327318403745899 ) ;
#30909=CARTESIAN_POINT ( 'NONE',  ( -2.050000000000032685, 2.500000000000000000, -6.495190528383302464 ) ) ;
#30910=ORIENTED_EDGE ( 'NONE', *, *, #117199, .T. ) ;
#30911=CARTESIAN_POINT ( 'NONE',  ( -8.550000000000011369, 2.500000000000000000, 1.718653347947321386 ) ) ;
#30912=CARTESIAN_POINT ( 'NONE',  ( 14.59999999999989484, 2.500000000000000000, -0.6928203230275541413 ) ) ;
#30913=EDGE_LOOP ( 'NONE', ( #43756, #37884 ) ) ;
#30914=CARTESIAN_POINT ( 'NONE',  ( -8.950000000000008171, 2.500000000000000000, 1.818653347947321475 ) ) ;
#30915=EDGE_CURVE ( 'NONE', #72308, #37406, #13731, .T. ) ;
#30916=VERTEX_POINT ( 'NONE', #115844 ) ;
#30917=DIRECTION ( 'NONE',  ( 0.000000000000000000, 1.000000000000000000, 0.000000000000000000 ) ) ;
#30918=VECTOR ( 'NONE', #125768, 1000.000000000000000 ) ;
#30919=CONICAL_SURFACE ( 'NONE', #85279, 0.1000000000000000472, 0.003490658503988666988 ) ;
#30920=VERTEX_POINT ( 'NONE', #5875 ) ;
#30921=LINE ( 'NONE', #72126, #121710 ) ;
#30922=FACE_OUTER_BOUND ( 'NONE', #33910, .T. ) ;
#30923=VERTEX_POINT ( 'NONE', #43267 ) ;
#30924=ADVANCED_FACE ( 'NONE', ( #63536 ), #45832, .T. ) ;
#30925=ORIENTED_EDGE ( 'NONE', *, *, #34103, .F. ) ;
#30926=DIRECTION ( 'NONE',  ( -4.274815082592931898E-19, -0.9999939076577903929, -0.003490651415223739937 ) ) ;
#30927=CARTESIAN_POINT ( 'NONE',  ( 2.699999999999944666, 12.50000000000000000, 4.676537180435972552 ) ) ;
#30928=EDGE_LOOP ( 'NONE', ( #10578, #33107, #84946, #9584 ) ) ;
#30929=VECTOR ( 'NONE', #36311, 1000.000000000000000 ) ;
#30930=LINE ( 'NONE', #72134, #74015 ) ;
#30932=VECTOR ( 'NONE', #52383, 1000.000000000000000 ) ;
#30933=CONICAL_SURFACE ( 'NONE', #53904, 0.09999999999999982514, 0.003490658503988666988 ) ;
#30934=CARTESIAN_POINT ( 'NONE',  ( -9.350000000000004974, 2.500000000000000000, 6.148780366869520897 ) ) ;
#30936=PLANE ( 'NONE',  #57221 ) ;
#30937=CARTESIAN_POINT ( 'NONE',  ( -2.900000000000030553, 2.500000000000000000, 4.922947341949748257 ) ) ;
#30938=CARTESIAN_POINT ( 'NONE',  ( 6.649999999999929301, 2.500000000000000000, 6.595190528383296780 ) ) ;
#30939=CIRCLE ( 'NONE', #47659, 0.06509327318403743123 ) ;
#30940=ORIENTED_EDGE ( 'NONE', *, *, #32285, .F. ) ;
#30941=EDGE_CURVE ( 'NONE', #91444, #19888, #85095, .T. ) ;
#30942=ORIENTED_EDGE ( 'NONE', *, *, #85848, .T. ) ;
#30943=FACE_OUTER_BOUND ( 'NONE', #115139, .T. ) ;
#30944=ORIENTED_EDGE ( 'NONE', *, *, #119268, .F. ) ;
#30945=CARTESIAN_POINT ( 'NONE',  ( -7.700000000000014388, 2.500000000000000000, -4.676537180435977881 ) ) ;
#30946=CARTESIAN_POINT ( 'NONE',  ( 9.149999999999916866, 12.50000000000000000, -2.857883832488653741 ) ) ;
#30947=DIRECTION ( 'NONE',  ( 0.000000000000000000, -0.000000000000000000, 1.000000000000000000 ) ) ;
#30948=ORIENTED_EDGE ( 'NONE', *, *, #7981, .F. ) ;
#30949=ORIENTED_EDGE ( 'NONE', *, *, #119262, .F. ) ;
#30950=FACE_BOUND ( 'NONE', #30380, .T. ) ;
#30951=VERTEX_POINT ( 'NONE', #4572 ) ;
#30952=DIRECTION ( 'NONE',  ( -0.000000000000000000, 1.000000000000000000, -0.000000000000000000 ) ) ;
#30953=DIRECTION ( 'NONE',  ( 0.000000000000000000, 1.000000000000000000, 0.000000000000000000 ) ) ;
#30954=ADVANCED_FACE ( 'NONE', ( #85735 ), #122424, .T. ) ;
#30955=DIRECTION ( 'NONE',  ( 0.000000000000000000, -0.9999939076577903929, 0.003490651415223739937 ) ) ;
#30956=ADVANCED_FACE ( 'NONE', ( #53705 ), #49268, .T. ) ;
#30957=AXIS2_PLACEMENT_3D ( 'NONE', #119259, #20428, #72114 ) ;
#30958=DIRECTION ( 'NONE',  ( -4.274815082592931898E-19, -0.9999939076577903929, -0.003490651415223739937 ) ) ;
#30959=CARTESIAN_POINT ( 'NONE',  ( 10.19999999999991047, 2.500000000000000000, -4.083716857408426826 ) ) ;
#30960=LINE ( 'NONE', #19840, #63216 ) ;
#30961=PLANE ( 'NONE',  #33031 ) ;
#30962=DIRECTION ( 'NONE',  ( 0.000000000000000000, 0.000000000000000000, 1.000000000000000000 ) ) ;
#30963=EDGE_CURVE ( 'NONE', #95802, #79005, #28327, .T. ) ;
#30964=EDGE_CURVE ( 'NONE', #114240, #98256, #5243, .T. ) ;
#30965=DIRECTION ( 'NONE',  ( 0.000000000000000000, 0.000000000000000000, -1.000000000000000000 ) ) ;
#30966=DIRECTION ( 'NONE',  ( 0.000000000000000000, 0.000000000000000000, -1.000000000000000000 ) ) ;
#30967=ADVANCED_FACE ( 'NONE', ( #53068 ), #5320, .T. ) ;
#30968=AXIS2_PLACEMENT_3D ( 'NONE', #87925, #95841, #38219 ) ;
#30969=EDGE_CURVE ( 'NONE', #5452, #40796, #125024, .T. ) ;
#30970=CIRCLE ( 'NONE', #106249, 0.1000000000000000472 ) ;
#30971=DIRECTION ( 'NONE',  ( 0.000000000000000000, 0.000000000000000000, 1.000000000000000000 ) ) ;
#30972=ORIENTED_EDGE ( 'NONE', *, *, #115253, .F. ) ;
#30973=CONICAL_SURFACE ( 'NONE', #99913, 0.1000000000000002554, 0.003490658503988666988 ) ;
#30974=ORIENTED_EDGE ( 'NONE', *, *, #84146, .T. ) ;
#30975=ORIENTED_EDGE ( 'NONE', *, *, #119183, .T. ) ;
#30976=EDGE_LOOP ( 'NONE', ( #101935, #40281 ) ) ;
#30977=LINE ( 'NONE', #90503, #95947 ) ;
#30978=EDGE_CURVE ( 'NONE', #23241, #17761, #116142, .T. ) ;
#30979=FACE_OUTER_BOUND ( 'NONE', #85509, .T. ) ;
#30980=EDGE_CURVE ( 'NONE', #86732, #113115, #80653, .T. ) ;
#30981=ORIENTED_EDGE ( 'NONE', *, *, #129498, .T. ) ;
#30982=VERTEX_POINT ( 'NONE', #39257 ) ;
#30983=VECTOR ( 'NONE', #93731, 1000.000000000000000 ) ;
#30984=VERTEX_POINT ( 'NONE', #7172 ) ;
#30986=EDGE_CURVE ( 'NONE', #47855, #6356, #97363, .T. ) ;
#30987=ADVANCED_FACE ( 'NONE', ( #6501 ), #18923, .T. ) ;
#30988=DIRECTION ( 'NONE',  ( 0.000000000000000000, 0.000000000000000000, 1.000000000000000000 ) ) ;
#30989=( LENGTH_UNIT ( ) NAMED_UNIT ( * ) SI_UNIT ( .MILLI., .METRE. ) );
#30990=DIRECTION ( 'NONE',  ( 0.000000000000000000, 0.000000000000000000, 1.000000000000000000 ) ) ;
#30991=DIRECTION ( 'NONE',  ( -4.274815082592931898E-19, -0.9999939076577903929, -0.003490651415223739937 ) ) ;
#30992=CARTESIAN_POINT ( 'NONE',  ( 2.500000000000001332, 2.392226903609812716, 9.521986658763283984 ) ) ;
#30993=CARTESIAN_POINT ( 'NONE',  ( -3.550000000000028244, 2.500000000000000000, 2.511473670974873507 ) ) ;
#30994=AXIS2_PLACEMENT_3D ( 'NONE', #51850, #77123, #29317 ) ;
#30996=ORIENTED_EDGE ( 'NONE', *, *, #111837, .T. ) ;
#30997=EDGE_CURVE ( 'NONE', #43893, #113036, #122228, .T. ) ;
#30998=ADVANCED_FACE ( 'NONE', ( #16336 ), #15592, .T. ) ;
#30999=CARTESIAN_POINT ( 'NONE',  ( -7.500000000000011546, 2.500000000000000000, 3.637306695894644726 ) ) ;
#31000=ORIENTED_EDGE ( 'NONE', *, *, #45383, .F. ) ;
#31001=AXIS2_PLACEMENT_3D ( 'NONE', #23407, #113746, #122279 ) ;
#31003=EDGE_LOOP ( 'NONE', ( #10142, #112066, #25083, #61723 ) ) ;
#31004=ORIENTED_EDGE ( 'NONE', *, *, #122758, .T. ) ;
#31005=LINE ( 'NONE', #41463, #81905 ) ;
#31006=ORIENTED_EDGE ( 'NONE', *, *, #108825, .T. ) ;
#31007=ORIENTED_EDGE ( 'NONE', *, *, #69193, .F. ) ;
#31008=EDGE_LOOP ( 'NONE', ( #69600, #31732 ) ) ;
#31009=CARTESIAN_POINT ( 'NONE',  ( -3.300000000000027800, 2.500000000000000000, -4.330127018922201643 ) ) ;
#31010=CARTESIAN_POINT ( 'NONE',  ( 4.549999999999937650, 12.50000000000000000, 2.165063509461097713 ) ) ;
#31011=DIRECTION ( 'NONE',  ( -0.000000000000000000, 1.000000000000000000, -0.000000000000000000 ) ) ;
#31012=DIRECTION ( 'NONE',  ( 0.000000000000000000, 0.000000000000000000, -1.000000000000000000 ) ) ;
#31013=DIRECTION ( 'NONE',  ( 0.000000000000000000, 1.000000000000000000, 0.000000000000000000 ) ) ;
#31014=CARTESIAN_POINT ( 'NONE',  ( 15.19999999999989271, 2.500000000000000000, -0.4464101615137783252 ) ) ;
#31015=DIRECTION ( 'NONE',  ( 0.000000000000000000, 1.000000000000000000, 0.000000000000000000 ) ) ;
#31016=VERTEX_POINT ( 'NONE', #26832 ) ;
#31017=CARTESIAN_POINT ( 'NONE',  ( 18.46077493895528931, 0.2575262203714444031, 4.048716073879469413 ) ) ;
#31018=VERTEX_POINT ( 'NONE', #77221 ) ;
#31020=CARTESIAN_POINT ( 'NONE',  ( 1.649999999999951950, 12.50000000000000000, -7.188010851410854052 ) ) ;
#31021=CIRCLE ( 'NONE', #83228, 0.1000000000000000472 ) ;
#31022=CIRCLE ( 'NONE', #47727, 0.1000000000000002554 ) ;
#31023=VERTEX_POINT ( 'NONE', #46455 ) ;
#31024=DIRECTION ( 'NONE',  ( 0.000000000000000000, 1.000000000000000000, 0.000000000000000000 ) ) ;
#31025=AXIS2_PLACEMENT_3D ( 'NONE', #29984, #109819, #7735 ) ;
#31026=CARTESIAN_POINT ( 'NONE',  ( -12.69999999999999396, 2.500000000000000000, -3.983716857408423628 ) ) ;
#31027=VERTEX_POINT ( 'NONE', #8454 ) ;
#31028=AXIS2_PLACEMENT_3D ( 'NONE', #66859, #17087, #57034 ) ;
#31029=EDGE_CURVE ( 'NONE', #16823, #116336, #122506, .T. ) ;
#31030=DIRECTION ( 'NONE',  ( -4.274815082592931898E-19, -0.9999939076577903929, -0.003490651415223739937 ) ) ;
#31031=EDGE_CURVE ( 'NONE', #30530, #94029, #11684, .T. ) ;
#31032=ORIENTED_EDGE ( 'NONE', *, *, #113563, .F. ) ;
#31033=ORIENTED_EDGE ( 'NONE', *, *, #67994, .F. ) ;
#31034=CARTESIAN_POINT ( 'NONE',  ( -13.34999999999999076, 12.50000000000000000, -2.099970236277062252 ) ) ;
#31035=DIRECTION ( 'NONE',  ( -0.000000000000000000, -1.000000000000000000, -0.000000000000000000 ) ) ;
#31037=PLANE ( 'NONE',  #128684 ) ;
#31038=CIRCLE ( 'NONE', #116676, 0.06509327318403745899 ) ;
#31039=ADVANCED_FACE ( 'NONE', ( #28121 ), #15881, .T. ) ;
#31040=DIRECTION ( 'NONE',  ( 0.000000000000000000, 0.000000000000000000, -1.000000000000000000 ) ) ;
#31041=VECTOR ( 'NONE', #92330, 1000.000000000000000 ) ;
#31042=ORIENTED_EDGE ( 'NONE', *, *, #92840, .F. ) ;
#31043=CARTESIAN_POINT ( 'NONE',  ( 1.649999999999950617, 2.500000000000000000, 2.265063509461097357 ) ) ;
#31044=ORIENTED_EDGE ( 'NONE', *, *, #111008, .F. ) ;
#31045=CARTESIAN_POINT ( 'NONE',  ( -14.79999999999998472, 2.500000000000000000, 0.3464101615137758494 ) ) ;
#31046=DIRECTION ( 'NONE',  ( 0.000000000000000000, 0.000000000000000000, -1.000000000000000000 ) ) ;
#31047=CONICAL_SURFACE ( 'NONE', #18488, 0.09999999999999982514, 0.003490658503988666988 ) ;
#31048=CIRCLE ( 'NONE', #85401, 0.06509327318403745899 ) ;
#31050=DIRECTION ( 'NONE',  ( -4.274815082592931898E-19, -0.9999939076577903929, -0.003490651415223739937 ) ) ;
#31051=CARTESIAN_POINT ( 'NONE',  ( -5.850000000000021849, 12.50000000000000000, -2.792790559304616504 ) ) ;
#31052=CARTESIAN_POINT ( 'NONE',  ( 2.299999999999949640, 2.500000000000000000, -0.2464101615137782308 ) ) ;
#31053=CARTESIAN_POINT ( 'NONE',  ( -4.350000000000023626, 2.500000000000000000, 6.841600689897072485 ) ) ;
#31054=VERTEX_POINT ( 'NONE', #18289 ) ;
#31055=AXIS2_PLACEMENT_3D ( 'NONE', #102000, #40521, #62086 ) ;
#31056=DIRECTION ( 'NONE',  ( 0.000000000000000000, 0.000000000000000000, 1.000000000000000000 ) ) ;
#31057=FACE_OUTER_BOUND ( 'NONE', #9316, .T. ) ;
#31058=CARTESIAN_POINT ( 'NONE',  ( 3.749999999999940492, 2.500000000000000000, 2.857883832488649301 ) ) ;
#31059=ORIENTED_EDGE ( 'NONE', *, *, #14386, .T. ) ;
#31060=AXIS2_PLACEMENT_3D ( 'NONE', #101168, #81527, #47722 ) ;
#31061=PLANE ( 'NONE',  #111705 ) ;
#31062=EDGE_CURVE ( 'NONE', #30982, #23344, #68108, .T. ) ;
#31063=AXIS2_PLACEMENT_3D ( 'NONE', #33467, #104744, #44563 ) ;
#31064=ORIENTED_EDGE ( 'NONE', *, *, #102143, .T. ) ;
#31065=ORIENTED_EDGE ( 'NONE', *, *, #115704, .T. ) ;
#31066=CARTESIAN_POINT ( 'NONE',  ( -9.200000000000009948, 2.500000000000000000, -4.330127018922197202 ) ) ;
#31067=ORIENTED_EDGE ( 'NONE', *, *, #12754, .T. ) ;
#31068=AXIS2_PLACEMENT_3D ( 'NONE', #7250, #95017, #45273 ) ;
#31069=CARTESIAN_POINT ( 'NONE',  ( 4.399999999999937295, 2.500000000000000000, 3.983716857408420964 ) ) ;
#31070=CARTESIAN_POINT ( 'NONE',  ( 6.249999999999968914, 2.500000000000000000, -6.495190528383302464 ) ) ;
#31071=EDGE_LOOP ( 'NONE', ( #105960, #18062, #53511, #125518 ) ) ;
#31072=CARTESIAN_POINT ( 'NONE',  ( 4.399999999999940847, 2.500000000000000000, -3.983716857408426293 ) ) ;
#31073=DIRECTION ( 'NONE',  ( -4.274815082592931898E-19, -0.9999939076577903929, -0.003490651415223739937 ) ) ;
#31074=ADVANCED_FACE ( 'NONE', ( #106668 ), #51425, .T. ) ;
#31075=CARTESIAN_POINT ( 'NONE',  ( 16.56576425165007294, -1.499999999999999778, -6.084390597445819893 ) ) ;
#31076=VECTOR ( 'NONE', #4985, 1000.000000000000000 ) ;
#31077=ORIENTED_EDGE ( 'NONE', *, *, #24178, .F. ) ;
#31078=CIRCLE ( 'NONE', #37334, 0.06509327318403745899 ) ;
#31079=CONICAL_SURFACE ( 'NONE', #104218, 0.1000000000000002554, 0.003490658503988666988 ) ;
#31080=ORIENTED_EDGE ( 'NONE', *, *, #59327, .F. ) ;
#31081=ORIENTED_EDGE ( 'NONE', *, *, #120757, .T. ) ;
#31082=DIRECTION ( 'NONE',  ( 0.000000000000000000, -0.000000000000000000, 1.000000000000000000 ) ) ;
#31083=CARTESIAN_POINT ( 'NONE',  ( 12.89999999999990266, 12.50000000000000000, 3.637306695894644726 ) ) ;
#31085=DIRECTION ( 'NONE',  ( 0.000000000000000000, 1.000000000000000000, 0.000000000000000000 ) ) ;
#31086=ADVANCED_FACE ( 'NONE', ( #27451 ), #84840, .T. ) ;
#31087=FACE_BOUND ( 'NONE', #96453, .T. ) ;
#31088=EDGE_LOOP ( 'NONE', ( #47608, #86328, #112867, #32781 ) ) ;
#31089=DIRECTION ( 'NONE',  ( 0.000000000000000000, 0.000000000000000000, -1.000000000000000000 ) ) ;
#31090=DIRECTION ( 'NONE',  ( 0.000000000000000000, -0.9999939076577903929, 0.003490651415223739937 ) ) ;
#31091=ORIENTED_EDGE ( 'NONE', *, *, #26783, .F. ) ;
#31092=DIRECTION ( 'NONE',  ( 0.000000000000000000, 0.000000000000000000, 1.000000000000000000 ) ) ;
#31093=CARTESIAN_POINT ( 'NONE',  ( -2.100000000000033840, 12.50000000000000000, 5.022947341949748790 ) ) ;
#31094=PLANE ( 'NONE',  #23545 ) ;
#31095=DIRECTION ( 'NONE',  ( 0.000000000000000000, -0.000000000000000000, 1.000000000000000000 ) ) ;
#31096=AXIS2_PLACEMENT_3D ( 'NONE', #100152, #90300, #10464 ) ;
#31097=CARTESIAN_POINT ( 'NONE',  ( 10.84999999999991260, 12.50000000000000000, -1.472243186433550122 ) ) ;
#31098=CARTESIAN_POINT ( 'NONE',  ( -8.150000000000012790, 2.500000000000000000, 2.511473670974873507 ) ) ;
#31099=CARTESIAN_POINT ( 'NONE',  ( 5.399999999999931966, 12.50000000000000000, 4.330127018922196314 ) ) ;
#31100=ORIENTED_EDGE ( 'NONE', *, *, #5205, .F. ) ;
#31101=VERTEX_POINT ( 'NONE', #56908 ) ;
#31102=AXIS2_PLACEMENT_3D ( 'NONE', #46257, #14210, #65896 ) ;
#31103=ORIENTED_EDGE ( 'NONE', *, *, #54810, .T. ) ;
#31104=EDGE_LOOP ( 'NONE', ( #38616, #15951 ) ) ;
#31105=LINE ( 'NONE', #71016, #47468 ) ;
#31106=DIRECTION ( 'NONE',  ( 0.000000000000000000, 0.000000000000000000, -1.000000000000000000 ) ) ;
#31107=VERTEX_POINT ( 'NONE', #88304 ) ;
#31108=FACE_BOUND ( 'NONE', #86519, .T. ) ;
#31109=FACE_OUTER_BOUND ( 'NONE', #7661, .T. ) ;
#31110=DIRECTION ( 'NONE',  ( 0.000000000000000000, 0.000000000000000000, -1.000000000000000000 ) ) ;
#31111=EDGE_CURVE ( 'NONE', #21032, #47772, #43115, .T. ) ;
#31112=CONICAL_SURFACE ( 'NONE', #35307, 0.1000000000000000056, 0.003490658503988666988 ) ;
#31113=CIRCLE ( 'NONE', #110511, 0.1000000000000000472 ) ;
#31114=DIRECTION ( 'NONE',  ( 0.000000000000000000, -0.9999939076577903929, 0.003490651415223739937 ) ) ;
#31115=CARTESIAN_POINT ( 'NONE',  ( 10.19999999999991047, 12.50000000000000000, -3.983716857408426293 ) ) ;
#31116=DIRECTION ( 'NONE',  ( -0.000000000000000000, -1.000000000000000000, -0.000000000000000000 ) ) ;
#31117=DIRECTION ( 'NONE',  ( 0.000000000000000000, -0.9999939076577903929, 0.003490651415223739937 ) ) ;
#31118=DIRECTION ( 'NONE',  ( -0.000000000000000000, 1.000000000000000000, -0.000000000000000000 ) ) ;
#31119=EDGE_CURVE ( 'NONE', #108711, #124173, #105779, .T. ) ;
#31120=LINE ( 'NONE', #3568, #97763 ) ;
#31121=ORIENTED_EDGE ( 'NONE', *, *, #98864, .T. ) ;
#31122=CONICAL_SURFACE ( 'NONE', #79227, 0.1000000000000002554, 0.003490658503988666988 ) ;
#31123=EDGE_CURVE ( 'NONE', #97390, #49498, #49065, .T. ) ;
#31124=VERTEX_POINT ( 'NONE', #19588 ) ;
#31125=ORIENTED_EDGE ( 'NONE', *, *, #114133, .F. ) ;
#31126=ORIENTED_EDGE ( 'NONE', *, *, #3610, .T. ) ;
#31127=EDGE_LOOP ( 'NONE', ( #82751, #26042 ) ) ;
#31128=ORIENTED_EDGE ( 'NONE', *, *, #5622, .F. ) ;
#31129=ADVANCED_FACE ( 'NONE', ( #70618 ), #88771, .T. ) ;
#31130=DIRECTION ( 'NONE',  ( 0.000000000000000000, 0.000000000000000000, 1.000000000000000000 ) ) ;
#31131=EDGE_CURVE ( 'NONE', #82531, #89806, #32367, .T. ) ;
#31132=EDGE_CURVE ( 'NONE', #94750, #41903, #39890, .T. ) ;
#31134=AXIS2_PLACEMENT_3D ( 'NONE', #119628, #50265, #40460 ) ;
#31135=CARTESIAN_POINT ( 'NONE',  ( 18.29531403502778986, 0.5011766475904848583, 4.780851392375770281 ) ) ;
#31136=ADVANCED_FACE ( 'NONE', ( #32000 ), #111841, .T. ) ;
#31137=CARTESIAN_POINT ( 'NONE',  ( 11.04999999999991189, 12.50000000000000000, -2.446380397790840266 ) ) ;
#31138=CARTESIAN_POINT ( 'NONE',  ( 3.749999999999942268, 2.500000000000000000, 1.372243186433545370 ) ) ;
#31139=FACE_OUTER_BOUND ( 'NONE', #26359, .T. ) ;
#31140=EDGE_LOOP ( 'NONE', ( #7211, #2626 ) ) ;
#31141=DIRECTION ( 'NONE',  ( 0.000000000000000000, 0.000000000000000000, 1.000000000000000000 ) ) ;
#31142=EDGE_CURVE ( 'NONE', #60850, #92191, #49080, .T. ) ;
#31143=ORIENTED_EDGE ( 'NONE', *, *, #108672, .T. ) ;
#31144=ORIENTED_EDGE ( 'NONE', *, *, #110924, .F. ) ;
#31145=VECTOR ( 'NONE', #128074, 1000.000000000000000 ) ;
#31146=DIRECTION ( 'NONE',  ( 0.000000000000000000, 0.000000000000000000, 1.000000000000000000 ) ) ;
#31147=CARTESIAN_POINT ( 'NONE',  ( 3.349999999999944578, 12.50000000000000000, -1.472243186433550122 ) ) ;
#31148=CARTESIAN_POINT ( 'NONE',  ( 12.69999999999990159, 2.500000000000000000, 4.676537180435972552 ) ) ;
#31149=EDGE_LOOP ( 'NONE', ( #126369, #68400, #105117, #16830 ) ) ;
#31150=AXIS2_PLACEMENT_3D ( 'NONE', #46108, #78160, #116772 ) ;
#31151=ORIENTED_EDGE ( 'NONE', *, *, #89792, .T. ) ;
#31152=FACE_OUTER_BOUND ( 'NONE', #34972, .T. ) ;
#31153=AXIS2_PLACEMENT_3D ( 'NONE', #79818, #49736, #120398 ) ;
#31154=CARTESIAN_POINT ( 'NONE',  ( -11.64999999999999680, 2.500000000000000000, 5.702370205355745014 ) ) ;
#31155=DIRECTION ( 'NONE',  ( 0.000000000000000000, 1.000000000000000000, 0.000000000000000000 ) ) ;
#31156=CARTESIAN_POINT ( 'NONE',  ( 9.149999999999915090, 2.500000000000000000, 6.395190528383296602 ) ) ;
#31157=VERTEX_POINT ( 'NONE', #11692 ) ;
#31158=DIRECTION ( 'NONE',  ( 0.000000000000000000, 0.000000000000000000, 1.000000000000000000 ) ) ;
#31159=CIRCLE ( 'NONE', #8137, 0.09999999999999982514 ) ;
#31160=ORIENTED_EDGE ( 'NONE', *, *, #95593, .F. ) ;
#31161=CARTESIAN_POINT ( 'NONE',  ( 10.63722763359394463, -2.500000000000000000, 8.014330155125172439 ) ) ;
#31162=EDGE_LOOP ( 'NONE', ( #17067, #50558, #58249, #1793 ) ) ;
#31163=DIRECTION ( 'NONE',  ( -0.000000000000000000, 1.000000000000000000, -0.000000000000000000 ) ) ;
#31164=CONICAL_SURFACE ( 'NONE', #49944, 0.09999999999999999167, 0.003490658503988666988 ) ;
#31165=VECTOR ( 'NONE', #80496, 1000.000000000000000 ) ;
#31166=CARTESIAN_POINT ( 'NONE',  ( -9.150000000000009237, 2.500000000000000000, 2.165063509461097713 ) ) ;
#31167=DIRECTION ( 'NONE',  ( 0.000000000000000000, 1.000000000000000000, 0.000000000000000000 ) ) ;
#31168=AXIS2_PLACEMENT_3D ( 'NONE', #37695, #47516, #87416 ) ;
#31169=DIRECTION ( 'NONE',  ( 0.000000000000000000, 0.000000000000000000, -1.000000000000000000 ) ) ;
#31170=ORIENTED_EDGE ( 'NONE', *, *, #100776, .T. ) ;
#31171=LINE ( 'NONE', #33108, #2853 ) ;
#31172=CIRCLE ( 'NONE', #20694, 0.1000000000000000056 ) ;
#31173=AXIS2_PLACEMENT_3D ( 'NONE', #42984, #102514, #103810 ) ;
#31174=EDGE_CURVE ( 'NONE', #16787, #57219, #2498, .T. ) ;
#31175=CARTESIAN_POINT ( 'NONE',  ( 2.049999999999950084, 2.500000000000000000, -2.165063509461101710 ) ) ;
#31176=ORIENTED_EDGE ( 'NONE', *, *, #103814, .T. ) ;
#31177=VERTEX_POINT ( 'NONE', #120372 ) ;
#31178=VERTEX_POINT ( 'NONE', #30065 ) ;
#31179=DIRECTION ( 'NONE',  ( -0.000000000000000000, 1.000000000000000000, -0.000000000000000000 ) ) ;
#31180=CARTESIAN_POINT ( 'NONE',  ( -10.85000000000000142, 12.50000000000000000, -5.802370205355746435 ) ) ;
#31181=CARTESIAN_POINT ( 'NONE',  ( -8.350000000000013856, 2.500000000000000000, -5.802370205355744659 ) ) ;
#31182=CARTESIAN_POINT ( 'NONE',  ( -2.300000000000032685, 2.500000000000000000, -0.2464101615137783419 ) ) ;
#31183=FACE_OUTER_BOUND ( 'NONE', #109577, .T. ) ;
#31185=EDGE_CURVE ( 'NONE', #62826, #57879, #21885, .T. ) ;
#31186=CARTESIAN_POINT ( 'NONE',  ( -10.65000000000000391, 12.50000000000000000, -6.148780366869522673 ) ) ;
#31187=DIRECTION ( 'NONE',  ( -0.000000000000000000, 1.000000000000000000, -0.000000000000000000 ) ) ;
#31188=CARTESIAN_POINT ( 'NONE',  ( 11.64999999999990443, 2.500000000000000000, -7.188010851410854052 ) ) ;
#31189=CIRCLE ( 'NONE', #112647, 0.06509327318403745899 ) ;
#31190=AXIS2_PLACEMENT_3D ( 'NONE', #45198, #55648, #94272 ) ;
#31191=AXIS2_PLACEMENT_3D ( 'NONE', #117103, #129555, #96827 ) ;
#31192=ORIENTED_EDGE ( 'NONE', *, *, #77282, .F. ) ;
#31193=CARTESIAN_POINT ( 'NONE',  ( 3.749999999999942268, 2.500000000000000000, -5.802370205355749988 ) ) ;
#31195=CARTESIAN_POINT ( 'NONE',  ( -1.250000000000037526, 2.500000000000000000, -1.372243186433550033 ) ) ;
#31196=CARTESIAN_POINT ( 'NONE',  ( -10.80000000000000249, 2.500000000000000000, -4.330127018922197202 ) ) ;
#31197=CONICAL_SURFACE ( 'NONE', #91822, 0.09999999999999982514, 0.003490658503988666988 ) ;
#31198=ORIENTED_EDGE ( 'NONE', *, *, #116091, .F. ) ;
#31199=CIRCLE ( 'NONE', #33355, 0.1000000000000002554 ) ;
#31200=CARTESIAN_POINT ( 'NONE',  ( -12.94999999999999218, 2.500000000000000000, 2.065063509461101621 ) ) ;
#31201=AXIS2_PLACEMENT_3D ( 'NONE', #106141, #86492, #25001 ) ;
#31202=DIRECTION ( 'NONE',  ( 0.000000000000000000, 0.000000000000000000, 1.000000000000000000 ) ) ;
#31203=CARTESIAN_POINT ( 'NONE',  ( 10.39999999999990976, 2.500000000000000000, -4.430127018922202176 ) ) ;
#31204=EDGE_LOOP ( 'NONE', ( #22952, #120389 ) ) ;
#31205=AXIS2_PLACEMENT_3D ( 'NONE', #26553, #57304, #48131 ) ;
#31206=ORIENTED_EDGE ( 'NONE', *, *, #1694, .T. ) ;
#31207=LINE ( 'NONE', #416, #38477 ) ;
#31208=AXIS2_PLACEMENT_3D ( 'NONE', #100079, #57586, #19581 ) ;
#31209=ADVANCED_FACE ( 'NONE', ( #111161 ), #22185, .T. ) ;
#31210=ORIENTED_EDGE ( 'NONE', *, *, #73494, .T. ) ;
#31211=ORIENTED_EDGE ( 'NONE', *, *, #113168, .F. ) ;
#31212=CARTESIAN_POINT ( 'NONE',  ( -12.29999999999999538, 2.500000000000000000, -4.576537180435975571 ) ) ;
#31213=CARTESIAN_POINT ( 'NONE',  ( 2.299999999999947864, 2.500000000000000000, 3.983716857408420964 ) ) ;
#31214=DIRECTION ( 'NONE',  ( 0.000000000000000000, 0.000000000000000000, 1.000000000000000000 ) ) ;
#31215=CARTESIAN_POINT ( 'NONE',  ( -2.950000000000029932, 2.500000000000000000, 2.265063509461097357 ) ) ;
#31216=ADVANCED_FACE ( 'NONE', ( #90901 ), #17948, .T. ) ;
#31217=ORIENTED_EDGE ( 'NONE', *, *, #7831, .T. ) ;
#31218=CARTESIAN_POINT ( 'NONE',  ( 1.899999999999951283, 12.50000000000000000, 0.4115034346978110880 ) ) ;
#31219=ORIENTED_EDGE ( 'NONE', *, *, #73652, .F. ) ;
#31220=CIRCLE ( 'NONE', #29168, 0.06509327318403745899 ) ;
#31221=EDGE_CURVE ( 'NONE', #39963, #13385, #21522, .T. ) ;
#31222=CARTESIAN_POINT ( 'NONE',  ( 12.69999999999990159, 12.50000000000000000, 4.676537180435972552 ) ) ;
#31224=ADVANCED_FACE ( 'NONE', ( #81716 ), #109910, .T. ) ;
#31225=ORIENTED_EDGE ( 'NONE', *, *, #65682, .F. ) ;
#31226=VERTEX_POINT ( 'NONE', #80450 ) ;
#31227=EDGE_CURVE ( 'NONE', #48633, #3662, #82527, .T. ) ;
#31228=ORIENTED_EDGE ( 'NONE', *, *, #20768, .T. ) ;
#31229=ORIENTED_EDGE ( 'NONE', *, *, #120359, .F. ) ;
#31230=DIRECTION ( 'NONE',  ( 0.000000000000000000, 0.000000000000000000, -1.000000000000000000 ) ) ;
#31231=CARTESIAN_POINT ( 'NONE',  ( 14.18215599412867967, 2.500000000000000000, 6.639800459772074781 ) ) ;
#31232=CARTESIAN_POINT ( 'NONE',  ( -9.600000000000008527, 12.50000000000000000, -3.637306695894645614 ) ) ;
#31233=EDGE_CURVE ( 'NONE', #16047, #21053, #45156, .T. ) ;
#31234=FACE_BOUND ( 'NONE', #8899, .T. ) ;
#31235=DIRECTION ( 'NONE',  ( -0.000000000000000000, 1.000000000000000000, -0.000000000000000000 ) ) ;
#31237=AXIS2_PLACEMENT_3D ( 'NONE', #72843, #63676, #83931 ) ;
#31238=CARTESIAN_POINT ( 'NONE',  ( 12.89999999999990266, 2.500000000000000000, -5.022947341949754119 ) ) ;
#31239=DIRECTION ( 'NONE',  ( 0.000000000000000000, 0.000000000000000000, 1.000000000000000000 ) ) ;
#31240=DIRECTION ( 'NONE',  ( 0.000000000000000000, 1.000000000000000000, 0.000000000000000000 ) ) ;
#31241=FACE_OUTER_BOUND ( 'NONE', #100622, .T. ) ;
#31242=VECTOR ( 'NONE', #8089, 1000.000000000000000 ) ;
#31244=CARTESIAN_POINT ( 'NONE',  ( 13.34999999999989662, 12.50000000000000000, -2.792790559304616504 ) ) ;
#31245=CIRCLE ( 'NONE', #93933, 0.06509327318403745899 ) ;
#31246=AXIS2_PLACEMENT_3D ( 'NONE', #88178, #66625, #105923 ) ;
#31247=ORIENTED_EDGE ( 'NONE', *, *, #12805, .T. ) ;
#31248=ORIENTED_EDGE ( 'NONE', *, *, #60668, .T. ) ;
#31249=ORIENTED_EDGE ( 'NONE', *, *, #97287, .F. ) ;
#31250=ORIENTED_EDGE ( 'NONE', *, *, #69688, .T. ) ;
#31251=VERTEX_POINT ( 'NONE', #89616 ) ;
#31252=DIRECTION ( 'NONE',  ( 0.000000000000000000, -0.9999939076577903929, 0.003490651415223739937 ) ) ;
#31253=AXIS2_PLACEMENT_3D ( 'NONE', #103705, #84040, #123968 ) ;
#31254=CARTESIAN_POINT ( 'NONE',  ( 4.349999999999941025, 12.50000000000000000, -1.883746621131363597 ) ) ;
#31255=ORIENTED_EDGE ( 'NONE', *, *, #103635, .T. ) ;
#31256=FACE_BOUND ( 'NONE', #120777, .T. ) ;
#31257=DIRECTION ( 'NONE',  ( -4.274815082592931898E-19, -0.9999939076577903929, -0.003490651415223739937 ) ) ;
#31258=VECTOR ( 'NONE', #120831, 1000.000000000000000 ) ;
#31259=AXIS2_PLACEMENT_3D ( 'NONE', #108309, #22372, #42661 ) ;
#31261=ORIENTED_EDGE ( 'NONE', *, *, #74403, .F. ) ;
#31262=DIRECTION ( 'NONE',  ( -0.000000000000000000, -1.000000000000000000, -0.000000000000000000 ) ) ;
#31263=DIRECTION ( 'NONE',  ( -0.000000000000000000, 1.000000000000000000, -0.000000000000000000 ) ) ;
#31264=CARTESIAN_POINT ( 'NONE',  ( -8.950000000000009948, 12.50000000000000000, 2.511473670974873507 ) ) ;
#31265=DIRECTION ( 'NONE',  ( 0.000000000000000000, 1.000000000000000000, 0.000000000000000000 ) ) ;
#31266=ORIENTED_EDGE ( 'NONE', *, *, #39790, .T. ) ;
#31268=EDGE_CURVE ( 'NONE', #109722, #69263, #129572, .T. ) ;
#31269=ORIENTED_EDGE ( 'NONE', *, *, #31896, .F. ) ;
#31270=EDGE_LOOP ( 'NONE', ( #107533, #16762 ) ) ;
#31271=AXIS2_PLACEMENT_3D ( 'NONE', #108513, #33670, #19486 ) ;
#31272=EDGE_CURVE ( 'NONE', #72904, #70366, #115957, .T. ) ;
#31273=PLANE ( 'NONE',  #25675 ) ;
#31274=CARTESIAN_POINT ( 'NONE',  ( 0.3999999999999563904, 12.50000000000000000, 5.022947341949748790 ) ) ;
#31275=ADVANCED_FACE ( 'NONE', ( #60801 ), #34701, .T. ) ;
#31276=ORIENTED_EDGE ( 'NONE', *, *, #117567, .F. ) ;
#31277=DIRECTION ( 'NONE',  ( -0.000000000000000000, -1.000000000000000000, -0.000000000000000000 ) ) ;
#31278=ADVANCED_FACE ( 'NONE', ( #64660 ), #33915, .T. ) ;
#31279=CIRCLE ( 'NONE', #41661, 0.1000000000000002554 ) ;
#31280=DIRECTION ( 'NONE',  ( 0.000000000000000000, 1.000000000000000000, 0.000000000000000000 ) ) ;
#31281=CARTESIAN_POINT ( 'NONE',  ( 11.24999999999990585, 12.50000000000000000, 2.922977105672686982 ) ) ;
#31282=FACE_OUTER_BOUND ( 'NONE', #112034, .T. ) ;
#31283=ADVANCED_FACE ( 'NONE', ( #12961 ), #22179, .T. ) ;
#31284=CARTESIAN_POINT ( 'NONE',  ( 7.099999999999928590, 2.500000000000000000, 3.737306695894644371 ) ) ;
#31285=ORIENTED_EDGE ( 'NONE', *, *, #111498, .F. ) ;
#31286=CONICAL_SURFACE ( 'NONE', #25011, 0.1000000000000000472, 0.003490658503988666988 ) ;
#31287=ORIENTED_EDGE ( 'NONE', *, *, #110865, .T. ) ;
#31288=CARTESIAN_POINT ( 'NONE',  ( 3.749999999999938716, 12.50000000000000000, 7.188010851410848723 ) ) ;
#31289=AXIS2_PLACEMENT_3D ( 'NONE', #105839, #26638, #88782 ) ;
#31290=AXIS2_PLACEMENT_3D ( 'NONE', #47885, #106776, #64920 ) ;
#31291=EDGE_CURVE ( 'NONE', #9874, #7088, #78606, .T. ) ;
#31292=CONICAL_SURFACE ( 'NONE', #41759, 0.09999999999999982514, 0.003490658503988666988 ) ;
#31293=EDGE_CURVE ( 'NONE', #71602, #10983, #112040, .T. ) ;
#31294=ORIENTED_EDGE ( 'NONE', *, *, #67463, .T. ) ;
#31295=DIRECTION ( 'NONE',  ( 0.000000000000000000, 0.000000000000000000, -1.000000000000000000 ) ) ;
#31296=ORIENTED_EDGE ( 'NONE', *, *, #78722, .F. ) ;
#31297=CARTESIAN_POINT ( 'NONE',  ( 8.949999999999921130, 12.50000000000000000, -6.841600689897078702 ) ) ;
#31298=DIRECTION ( 'NONE',  ( -0.000000000000000000, 1.000000000000000000, -0.000000000000000000 ) ) ;
#31299=DIRECTION ( 'NONE',  ( -0.000000000000000000, 1.000000000000000000, -0.000000000000000000 ) ) ;
#31300=CARTESIAN_POINT ( 'NONE',  ( 7.299999999999927880, 12.50000000000000000, 3.983716857408420964 ) ) ;
#31301=CARTESIAN_POINT ( 'NONE',  ( -2.900000000000029221, 2.500000000000000000, -0.6928203230275541413 ) ) ;
#31302=AXIS2_PLACEMENT_3D ( 'NONE', #116058, #108804, #95779 ) ;
#31303=VERTEX_POINT ( 'NONE', #34583 ) ;
#31304=ORIENTED_EDGE ( 'NONE', *, *, #89150, .T. ) ;
#31305=VECTOR ( 'NONE', #107652, 1000.000000000000000 ) ;
#31306=EDGE_LOOP ( 'NONE', ( #123909, #26273, #58901, #67012 ) ) ;
#31307=DIRECTION ( 'NONE',  ( -4.274815082592931898E-19, -0.9999939076577903929, -0.003490651415223739937 ) ) ;
#31308=AXIS2_PLACEMENT_3D ( 'NONE', #35565, #56466, #4779 ) ;
#31309=CARTESIAN_POINT ( 'NONE',  ( -8.350000000000012079, 12.50000000000000000, 2.857883832488649301 ) ) ;
#31310=DIRECTION ( 'NONE',  ( -0.000000000000000000, 1.000000000000000000, -0.000000000000000000 ) ) ;
#31311=EDGE_LOOP ( 'NONE', ( #56189, #42871, #62316, #4818 ) ) ;
#31312=ORIENTED_EDGE ( 'NONE', *, *, #70349, .T. ) ;
#31313=EDGE_LOOP ( 'NONE', ( #71876, #98117, #36453, #108310 ) ) ;
#31314=FACE_OUTER_BOUND ( 'NONE', #52595, .T. ) ;
#31315=ORIENTED_EDGE ( 'NONE', *, *, #34949, .F. ) ;
#31316=DIRECTION ( 'NONE',  ( -0.000000000000000000, 1.000000000000000000, -0.000000000000000000 ) ) ;
#31317=DIRECTION ( 'NONE',  ( 0.000000000000000000, -0.9999939076577903929, 0.003490651415223739937 ) ) ;
#31318=CARTESIAN_POINT ( 'NONE',  ( -1.450000000000035927, 12.50000000000000000, -6.148780366869526226 ) ) ;
#31319=DIRECTION ( 'NONE',  ( 0.000000000000000000, 0.000000000000000000, 1.000000000000000000 ) ) ;
#31321=LINE ( 'NONE', #19544, #73416 ) ;
#31322=AXIS2_PLACEMENT_3D ( 'NONE', #90512, #108224, #59142 ) ;
#31323=CARTESIAN_POINT ( 'NONE',  ( 10.44999999999991402, 12.50000000000000000, 6.495190528383297135 ) ) ;
#31324=DIRECTION ( 'NONE',  ( 0.000000000000000000, -0.000000000000000000, 1.000000000000000000 ) ) ;
#31325=EDGE_LOOP ( 'NONE', ( #59669, #22631, #97937, #108847 ) ) ;
#31326=DIRECTION ( 'NONE',  ( 0.000000000000000000, 1.000000000000000000, 0.000000000000000000 ) ) ;
#31327=DIRECTION ( 'NONE',  ( 0.000000000000000000, 0.000000000000000000, 1.000000000000000000 ) ) ;
#31328=ORIENTED_EDGE ( 'NONE', *, *, #56724, .T. ) ;
#31329=ORIENTED_EDGE ( 'NONE', *, *, #81856, .F. ) ;
#31332=LINE ( 'NONE', #62721, #126338 ) ;
#31333=DIRECTION ( 'NONE',  ( 0.000000000000000000, -0.9999939076577903929, 0.003490651415223739937 ) ) ;
#31334=CARTESIAN_POINT ( 'NONE',  ( -11.05000000000000071, 2.500000000000000000, 6.841600689897072485 ) ) ;
#31335=CARTESIAN_POINT ( 'NONE',  ( 13.14999999999990088, 12.50000000000000000, 1.753560074763284016 ) ) ;
#31336=EDGE_CURVE ( 'NONE', #47870, #126052, #126430, .T. ) ;
#31338=DIRECTION ( 'NONE',  ( 0.000000000000000000, 0.000000000000000000, 1.000000000000000000 ) ) ;
#31339=DIRECTION ( 'NONE',  ( -4.274815082592931898E-19, -0.9999939076577903929, -0.003490651415223739937 ) ) ;
#31340=CIRCLE ( 'NONE', #71115, 0.06509327318403741736 ) ;
#31341=CARTESIAN_POINT ( 'NONE',  ( 12.89999999999990088, 12.50000000000000000, 4.395220292106234439 ) ) ;
#31342=VERTEX_POINT ( 'NONE', #65290 ) ;
#31343=ORIENTED_EDGE ( 'NONE', *, *, #86361, .F. ) ;
#31344=VECTOR ( 'NONE', #36357, 1000.000000000000000 ) ;
#31345=ORIENTED_EDGE ( 'NONE', *, *, #9637, .T. ) ;
#31346=CIRCLE ( 'NONE', #39482, 0.1000000000000002554 ) ;
#31347=EDGE_LOOP ( 'NONE', ( #4518, #30794, #107578, #46100 ) ) ;
#31348=ORIENTED_EDGE ( 'NONE', *, *, #94664, .F. ) ;
#31349=CARTESIAN_POINT ( 'NONE',  ( -10.40000000000000213, 2.500000000000000000, 3.537306695894645081 ) ) ;
#31350=DIRECTION ( 'NONE',  ( 0.000000000000000000, 0.000000000000000000, 1.000000000000000000 ) ) ;
#31351=CIRCLE ( 'NONE', #58543, 0.1000000000000002554 ) ;
#31352=AXIS2_PLACEMENT_3D ( 'NONE', #57621, #37344, #79203 ) ;
#31353=ORIENTED_EDGE ( 'NONE', *, *, #10766, .T. ) ;
#31354=CARTESIAN_POINT ( 'NONE',  ( 11.04999999999991189, 2.500000000000000000, -2.611473670974877592 ) ) ;
#31355=CARTESIAN_POINT ( 'NONE',  ( 9.199999999999915801, 2.500000000000000000, -4.330127018922201643 ) ) ;
#31356=DIRECTION ( 'NONE',  ( 0.000000000000000000, 0.000000000000000000, -1.000000000000000000 ) ) ;
#31357=DIRECTION ( 'NONE',  ( 0.000000000000000000, 0.000000000000000000, 1.000000000000000000 ) ) ;
#31358=ORIENTED_EDGE ( 'NONE', *, *, #5389, .T. ) ;
#31359=DIRECTION ( 'NONE',  ( 0.000000000000000000, 0.000000000000000000, -1.000000000000000000 ) ) ;
#31360=DIRECTION ( 'NONE',  ( 0.000000000000000000, 0.000000000000000000, 1.000000000000000000 ) ) ;
#31361=VERTEX_POINT ( 'NONE', #123567 ) ;
#31362=ORIENTED_EDGE ( 'NONE', *, *, #46216, .T. ) ;
#31363=ORIENTED_EDGE ( 'NONE', *, *, #65789, .F. ) ;
#31364=VERTEX_POINT ( 'NONE', #94765 ) ;
#31365=DIRECTION ( 'NONE',  ( 0.000000000000000000, -0.000000000000000000, 1.000000000000000000 ) ) ;
#31366=CARTESIAN_POINT ( 'NONE',  ( 5.399999999999934630, 2.500000000000000000, -0.7928203230275543412 ) ) ;
#31367=DIRECTION ( 'NONE',  ( -0.000000000000000000, 1.000000000000000000, -0.000000000000000000 ) ) ;
#31368=AXIS2_PLACEMENT_3D ( 'NONE', #123912, #119191, #1338 ) ;
#31369=ADVANCED_FACE ( 'NONE', ( #73840 ), #74486, .T. ) ;
#31370=EDGE_LOOP ( 'NONE', ( #31065, #40153 ) ) ;
#31371=LINE ( 'NONE', #112504, #56477 ) ;
#31372=VERTEX_POINT ( 'NONE', #113773 ) ;
#31373=LINE ( 'NONE', #58893, #28683 ) ;
#31374=CARTESIAN_POINT ( 'NONE',  ( 17.91370874550471370, -0.4812889678260146020, -4.985910759330065112 ) ) ;
#31375=ADVANCED_FACE ( 'NONE', ( #105229 ), #64021, .T. ) ;
#31376=DIRECTION ( 'NONE',  ( 0.000000000000000000, 1.000000000000000000, 0.000000000000000000 ) ) ;
#31377=CARTESIAN_POINT ( 'NONE',  ( 6.449999999999930012, 2.500000000000000000, -1.818653347947326138 ) ) ;
#31378=ADVANCED_FACE ( 'NONE', ( #24743 ), #61684, .T. ) ;
#31379=AXIS2_PLACEMENT_3D ( 'NONE', #104600, #5106, #124894 ) ;
#31380=ORIENTED_EDGE ( 'NONE', *, *, #170, .F. ) ;
#31381=VERTEX_POINT ( 'NONE', #14262 ) ;
#31382=EDGE_CURVE ( 'NONE', #7675, #60793, #86711, .T. ) ;
#31383=EDGE_CURVE ( 'NONE', #111448, #24152, #15544, .T. ) ;
#31384=EDGE_LOOP ( 'NONE', ( #100715, #123638 ) ) ;
#31385=DIRECTION ( 'NONE',  ( 0.000000000000000000, -0.9999939076577903929, 0.003490651415223739937 ) ) ;
#31386=ADVANCED_FACE ( 'NONE', ( #4420 ), #105590, .T. ) ;
#31387=DIRECTION ( 'NONE',  ( 0.000000000000000000, 0.000000000000000000, 1.000000000000000000 ) ) ;
#31388=ADVANCED_FACE ( 'NONE', ( #102647 ), #80471, .T. ) ;
#31389=FACE_BOUND ( 'NONE', #105783, .T. ) ;
#31390=AXIS2_PLACEMENT_3D ( 'NONE', #69213, #125706, #68575 ) ;
#31391=FACE_OUTER_BOUND ( 'NONE', #49198, .T. ) ;
#31392=DIRECTION ( 'NONE',  ( 0.000000000000000000, 1.000000000000000000, 0.000000000000000000 ) ) ;
#31393=CARTESIAN_POINT ( 'NONE',  ( -12.09999999999999609, 2.500000000000000000, -4.922947341949750921 ) ) ;
#31394=AXIS2_PLACEMENT_3D ( 'NONE', #2188, #72877, #46635 ) ;
#31395=AXIS2_PLACEMENT_3D ( 'NONE', #113961, #24290, #124428 ) ;
#31396=CARTESIAN_POINT ( 'NONE',  ( 10.39999999999991154, 12.50000000000000000, 5.022947341949748790 ) ) ;
#31398=PLANE ( 'NONE',  #46959 ) ;
#31399=ORIENTED_EDGE ( 'NONE', *, *, #30374, .F. ) ;
#31400=CIRCLE ( 'NONE', #114899, 0.09999999999999982514 ) ;
#31401=LINE ( 'NONE', #30765, #76222 ) ;
#31402=DIRECTION ( 'NONE',  ( -0.000000000000000000, -1.000000000000000000, -0.000000000000000000 ) ) ;
#31403=AXIS2_PLACEMENT_3D ( 'NONE', #39936, #111891, #89669 ) ;
#31404=ORIENTED_EDGE ( 'NONE', *, *, #26052, .F. ) ;
#31405=VERTEX_POINT ( 'NONE', #3175 ) ;
#31406=PLANE ( 'NONE',  #117131 ) ;
#31407=CARTESIAN_POINT ( 'NONE',  ( -6.050000000000022027, 2.500000000000000000, -6.048780366869526581 ) ) ;
#31408=FACE_BOUND ( 'NONE', #24483, .T. ) ;
#31409=DIRECTION ( 'NONE',  ( 0.000000000000000000, 1.000000000000000000, 0.000000000000000000 ) ) ;
#31410=ORIENTED_EDGE ( 'NONE', *, *, #28841, .F. ) ;
#31411=DIRECTION ( 'NONE',  ( 0.000000000000000000, 1.000000000000000000, 0.000000000000000000 ) ) ;
#31412=EDGE_CURVE ( 'NONE', #48527, #55655, #43122, .T. ) ;
#31414=ORIENTED_EDGE ( 'NONE', *, *, #234, .F. ) ;
#31415=CARTESIAN_POINT ( 'NONE',  ( -4.350000000000023626, 2.500000000000000000, -2.511473670974877948 ) ) ;
#31416=CARTESIAN_POINT ( 'NONE',  ( 13.54999999999989768, 2.500000000000000000, -2.411473670974877859 ) ) ;
#31417=AXIS2_PLACEMENT_3D ( 'NONE', #114834, #66390, #33711 ) ;
#31418=EDGE_CURVE ( 'NONE', #105096, #106661, #24022, .T. ) ;
#31419=EDGE_CURVE ( 'NONE', #30923, #115271, #72141, .T. ) ;
#31420=CARTESIAN_POINT ( 'NONE',  ( -11.64999999999999680, 12.50000000000000000, -2.857883832488649745 ) ) ;
#31421=CARTESIAN_POINT ( 'NONE',  ( -11.84999999999999787, 12.50000000000000000, -6.148780366869522673 ) ) ;
#31422=EDGE_CURVE ( 'NONE', #106999, #30477, #21983, .T. ) ;
#31423=EDGE_LOOP ( 'NONE', ( #106706, #110305, #88755, #95240 ) ) ;
#31424=CARTESIAN_POINT ( 'NONE',  ( 2.899999999999946620, 12.50000000000000000, -3.637306695894650055 ) ) ;
#31426=DIRECTION ( 'NONE',  ( 0.000000000000000000, 0.000000000000000000, 1.000000000000000000 ) ) ;
#31427=CARTESIAN_POINT ( 'NONE',  ( -12.09999999999999609, 2.500000000000000000, 4.230127018922196669 ) ) ;
#31428=EDGE_CURVE ( 'NONE', #93141, #22544, #69996, .T. ) ;
#31429=VERTEX_POINT ( 'NONE', #35852 ) ;
#31430=ORIENTED_EDGE ( 'NONE', *, *, #16427, .T. ) ;
#31431=EDGE_CURVE ( 'NONE', #356, #22999, #11497, .T. ) ;
#31432=DIRECTION ( 'NONE',  ( 0.000000000000000000, 0.000000000000000000, -1.000000000000000000 ) ) ;
#31433=EDGE_CURVE ( 'NONE', #91784, #68041, #1030, .T. ) ;
#31434=ORIENTED_EDGE ( 'NONE', *, *, #77105, .F. ) ;
#31435=DIRECTION ( 'NONE',  ( 0.000000000000000000, 0.000000000000000000, 1.000000000000000000 ) ) ;
#31436=DIRECTION ( 'NONE',  ( -4.274815082592931898E-19, -0.9999939076577903929, -0.003490651415223739937 ) ) ;
#31437=EDGE_CURVE ( 'NONE', #119726, #85603, #106516, .T. ) ;
#31438=ADVANCED_FACE ( 'NONE', ( #97983 ), #47015, .T. ) ;
#31439=DIRECTION ( 'NONE',  ( -0.000000000000000000, -1.000000000000000000, -0.000000000000000000 ) ) ;
#31440=ORIENTED_EDGE ( 'NONE', *, *, #2633, .T. ) ;
#31441=DIRECTION ( 'NONE',  ( -0.000000000000000000, 1.000000000000000000, -0.000000000000000000 ) ) ;
#31442=DIRECTION ( 'NONE',  ( -0.000000000000000000, -1.000000000000000000, -0.000000000000000000 ) ) ;
#31443=CARTESIAN_POINT ( 'NONE',  ( 4.399999999999937295, 2.500000000000000000, 4.676537180435972552 ) ) ;
#31444=CARTESIAN_POINT ( 'NONE',  ( -5.400000000000019895, 2.500000000000000000, -2.276824562219559311E-15 ) ) ;
#31445=CARTESIAN_POINT ( 'NONE',  ( -4.119968255444916849E-14, 12.50000000000000000, 3.702399969078682407 ) ) ;
#31446=DIRECTION ( 'NONE',  ( 0.000000000000000000, 1.000000000000000000, 0.000000000000000000 ) ) ;
#31447=EDGE_CURVE ( 'NONE', #27262, #106163, #90917, .T. ) ;
#31448=ORIENTED_EDGE ( 'NONE', *, *, #13774, .F. ) ;
#31449=ORIENTED_EDGE ( 'NONE', *, *, #120038, .T. ) ;
#31450=CARTESIAN_POINT ( 'NONE',  ( -6.650000000000014566, 2.500000000000000000, 2.265063509461097357 ) ) ;
#31451=EDGE_LOOP ( 'NONE', ( #100218, #83883, #82812, #60554 ) ) ;
#31452=FACE_OUTER_BOUND ( 'NONE', #120312, .T. ) ;
#31453=ORIENTED_EDGE ( 'NONE', *, *, #16592, .F. ) ;
#31454=ORIENTED_EDGE ( 'NONE', *, *, #9953, .T. ) ;
#31455=ORIENTED_EDGE ( 'NONE', *, *, #32287, .T. ) ;
#31456=DIRECTION ( 'NONE',  ( 0.000000000000000000, 0.000000000000000000, 1.000000000000000000 ) ) ;
#31457=AXIS2_PLACEMENT_3D ( 'NONE', #34032, #124987, #15655 ) ;
#31458=CARTESIAN_POINT ( 'NONE',  ( 11.64999999999990266, 12.50000000000000000, 2.165063509461097713 ) ) ;
#31459=CIRCLE ( 'NONE', #64875, 0.06509327318403745899 ) ;
#31460=DIRECTION ( 'NONE',  ( 0.000000000000000000, 0.000000000000000000, 1.000000000000000000 ) ) ;
#31461=FACE_OUTER_BOUND ( 'NONE', #91160, .T. ) ;
#31462=CARTESIAN_POINT ( 'NONE',  ( 2.699999999999947331, 2.500000000000000000, -0.3464101615137783474 ) ) ;
#31463=CARTESIAN_POINT ( 'NONE',  ( 2.899999999999943956, 2.500000000000000000, 4.330127018922196314 ) ) ;
#31464=DIRECTION ( 'NONE',  ( -0.000000000000000000, -1.000000000000000000, -0.000000000000000000 ) ) ;
#31465=CARTESIAN_POINT ( 'NONE',  ( 4.149999999999939959, 2.500000000000000000, 2.957883832488649389 ) ) ;
#31466=CARTESIAN_POINT ( 'NONE',  ( 6.899999999999928413, 2.500000000000000000, -4.776537180435977525 ) ) ;
#31467=AXIS2_PLACEMENT_3D ( 'NONE', #123593, #113792, #65309 ) ;
#31468=VERTEX_POINT ( 'NONE', #45679 ) ;
#31469=DIRECTION ( 'NONE',  ( -0.000000000000000000, -1.000000000000000000, -0.000000000000000000 ) ) ;
#31470=ORIENTED_EDGE ( 'NONE', *, *, #96294, .T. ) ;
#31471=ORIENTED_EDGE ( 'NONE', *, *, #97045, .F. ) ;
#31473=DIRECTION ( 'NONE',  ( 0.000000000000000000, 1.000000000000000000, 0.000000000000000000 ) ) ;
#31474=CIRCLE ( 'NONE', #94160, 0.06509327318403743123 ) ;
#31475=CARTESIAN_POINT ( 'NONE',  ( -8.350000000000012079, 2.500000000000000000, 2.857883832488649301 ) ) ;
#31476=AXIS2_PLACEMENT_3D ( 'NONE', #56150, #74522, #54859 ) ;
#31477=EDGE_CURVE ( 'NONE', #128465, #102223, #84653, .T. ) ;
#31478=DIRECTION ( 'NONE',  ( 0.000000000000000000, 0.000000000000000000, -1.000000000000000000 ) ) ;
#31479=DIRECTION ( 'NONE',  ( -4.274815082592931898E-19, -0.9999939076577903929, -0.003490651415223739937 ) ) ;
#31480=CARTESIAN_POINT ( 'NONE',  ( -10.84999999999999964, 2.500000000000000000, 5.802370205355744659 ) ) ;
#31481=VERTEX_POINT ( 'NONE', #57429 ) ;
#31482=AXIS2_PLACEMENT_3D ( 'NONE', #28151, #68065, #58904 ) ;
#31483=ORIENTED_EDGE ( 'NONE', *, *, #4062, .T. ) ;
#31484=VERTEX_POINT ( 'NONE', #27299 ) ;
#31485=CARTESIAN_POINT ( 'NONE',  ( 9.399999999999915090, 12.50000000000000000, 4.676537180435972552 ) ) ;
#31486=AXIS2_PLACEMENT_3D ( 'NONE', #26569, #117487, #13008 ) ;
#31487=VERTEX_POINT ( 'NONE', #108445 ) ;
#31489=EDGE_LOOP ( 'NONE', ( #25575, #98938 ) ) ;
#31490=CARTESIAN_POINT ( 'NONE',  ( -8.350000000000013856, 12.50000000000000000, -6.495190528383297135 ) ) ;
#31491=CARTESIAN_POINT ( 'NONE',  ( -4.999999999999990230, 2.500000000000000000, -4.330127018922201643 ) ) ;
#31492=DIRECTION ( 'NONE',  ( -0.000000000000000000, 1.000000000000000000, -0.000000000000000000 ) ) ;
#31493=DIRECTION ( 'NONE',  ( 0.000000000000000000, 0.000000000000000000, 1.000000000000000000 ) ) ;
#31494=LINE ( 'NONE', #92333, #30498 ) ;
#31495=ORIENTED_EDGE ( 'NONE', *, *, #91366, .T. ) ;
#31496=DIRECTION ( 'NONE',  ( 0.000000000000000000, 0.000000000000000000, 1.000000000000000000 ) ) ;
#31497=DIRECTION ( 'NONE',  ( -0.000000000000000000, 1.000000000000000000, -0.000000000000000000 ) ) ;
#31498=DIRECTION ( 'NONE',  ( -0.000000000000000000, 1.000000000000000000, -0.000000000000000000 ) ) ;
#31499=DIRECTION ( 'NONE',  ( -0.000000000000000000, -1.000000000000000000, -0.000000000000000000 ) ) ;
#31500=DIRECTION ( 'NONE',  ( -0.000000000000000000, 1.000000000000000000, -0.000000000000000000 ) ) ;
#31501=EDGE_LOOP ( 'NONE', ( #10130, #53097, #114971, #20158 ) ) ;
#31502=EDGE_LOOP ( 'NONE', ( #127875, #63466 ) ) ;
#31503=ORIENTED_EDGE ( 'NONE', *, *, #28908, .F. ) ;
#31504=VECTOR ( 'NONE', #98261, 1000.000000000000000 ) ;
#31505=CARTESIAN_POINT ( 'NONE',  ( -11.69999999999999929, 12.50000000000000000, -4.330127018922198978 ) ) ;
#31506=VECTOR ( 'NONE', #95719, 1000.000000000000000 ) ;
#31507=CIRCLE ( 'NONE', #94194, 7.500000000000000000 ) ;
#31508=EDGE_LOOP ( 'NONE', ( #53148, #99493, #65596, #3996 ) ) ;
#31509=CARTESIAN_POINT ( 'NONE',  ( -2.100000000000033840, 2.500000000000000000, 5.122947341949749323 ) ) ;
#31510=DIRECTION ( 'NONE',  ( 0.000000000000000000, 0.000000000000000000, 1.000000000000000000 ) ) ;
#31511=ADVANCED_FACE ( 'NONE', ( #97345 ), #7659, .T. ) ;
#31512=AXIS2_PLACEMENT_3D ( 'NONE', #1402, #41357, #81265 ) ;
#31513=AXIS2_PLACEMENT_3D ( 'NONE', #81522, #121429, #102450 ) ;
#31514=ORIENTED_EDGE ( 'NONE', *, *, #110352, .F. ) ;
#31515=LINE ( 'NONE', #30890, #7641 ) ;
#31516=DIRECTION ( 'NONE',  ( -0.000000000000000000, 1.000000000000000000, -0.000000000000000000 ) ) ;
#31517=CARTESIAN_POINT ( 'NONE',  ( 2.699999999999946443, 2.500000000000000000, -3.883716857408426648 ) ) ;
#31518=LINE ( 'NONE', #101549, #95752 ) ;
#31519=EDGE_CURVE ( 'NONE', #71951, #97815, #105877, .T. ) ;
#31520=DIRECTION ( 'NONE',  ( 0.000000000000000000, -0.9999939076577903929, 0.003490651415223739937 ) ) ;
#31521=ORIENTED_EDGE ( 'NONE', *, *, #2053, .F. ) ;
#31522=ADVANCED_FACE ( 'NONE', ( #117596 ), #38718, .T. ) ;
#31523=EDGE_CURVE ( 'NONE', #65236, #125999, #109793, .T. ) ;
#31524=EDGE_LOOP ( 'NONE', ( #128414, #62809, #2246, #107014 ) ) ;
#31526=CARTESIAN_POINT ( 'NONE',  ( 35.03127169446342037, 3.271239217524853249, -3.345729450120381365 ) ) ;
#31527=EDGE_CURVE ( 'NONE', #15198, #122612, #18776, .T. ) ;
#31529=DIRECTION ( 'NONE',  ( -4.274815082592931898E-19, -0.9999939076577903929, -0.003490651415223739937 ) ) ;
#31530=FACE_OUTER_BOUND ( 'NONE', #21649, .T. ) ;
#31531=LINE ( 'NONE', #71433, #91885 ) ;
#31532=VERTEX_POINT ( 'NONE', #48907 ) ;
#31533=ORIENTED_EDGE ( 'NONE', *, *, #14929, .F. ) ;
#31534=CARTESIAN_POINT ( 'NONE',  ( -11.84999999999999787, 2.500000000000000000, -2.511473670974873951 ) ) ;
#31535=DIRECTION ( 'NONE',  ( 0.000000000000000000, 1.000000000000000000, 0.000000000000000000 ) ) ;
#31536=EDGE_CURVE ( 'NONE', #2251, #113231, #57474, .T. ) ;
#31537=CARTESIAN_POINT ( 'NONE',  ( -11.44999999999999751, 12.50000000000000000, 6.213873640053559022 ) ) ;
#31538=DIRECTION ( 'NONE',  ( 0.000000000000000000, -0.000000000000000000, 1.000000000000000000 ) ) ;
#31539=ORIENTED_EDGE ( 'NONE', *, *, #68407, .T. ) ;
#31540=EDGE_CURVE ( 'NONE', #86369, #39107, #42920, .T. ) ;
#31541=CONICAL_SURFACE ( 'NONE', #50323, 0.1000000000000002554, 0.003490658503988666988 ) ;
#31542=DIRECTION ( 'NONE',  ( 0.000000000000000000, 0.000000000000000000, 1.000000000000000000 ) ) ;
#31543=EDGE_CURVE ( 'NONE', #66987, #92109, #44954, .T. ) ;
#31544=AXIS2_PLACEMENT_3D ( 'NONE', #128733, #68484, #8908 ) ;
#31545=DIRECTION ( 'NONE',  ( 0.000000000000000000, 1.000000000000000000, 0.000000000000000000 ) ) ;
#31546=VERTEX_POINT ( 'NONE', #91385 ) ;
#31547=FACE_OUTER_BOUND ( 'NONE', #99871, .T. ) ;
#31548=ORIENTED_EDGE ( 'NONE', *, *, #39539, .F. ) ;
#31549=AXIS2_PLACEMENT_3D ( 'NONE', #8329, #48263, #39120 ) ;
#31550=DIRECTION ( 'NONE',  ( -4.274815082592931898E-19, -0.9999939076577903929, -0.003490651415223739937 ) ) ;
#31551=AXIS2_PLACEMENT_3D ( 'NONE', #13096, #123077, #54331 ) ;
#31552=ORIENTED_EDGE ( 'NONE', *, *, #50024, .T. ) ;
#31553=ORIENTED_EDGE ( 'NONE', *, *, #25295, .T. ) ;
#31554=DIRECTION ( 'NONE',  ( 0.000000000000000000, 1.000000000000000000, 0.000000000000000000 ) ) ;
#31555=CARTESIAN_POINT ( 'NONE',  ( 10.61495711629421557, 2.499999999999999112, -8.020491763388227113 ) ) ;
#31556=VERTEX_POINT ( 'NONE', #22027 ) ;
#31557=EDGE_LOOP ( 'NONE', ( #22003, #65006, #94542, #58272 ) ) ;
#31558=DIRECTION ( 'NONE',  ( -4.274815082592931898E-19, -0.9999939076577903929, -0.003490651415223739937 ) ) ;
#31559=DIRECTION ( 'NONE',  ( 0.000000000000000000, 0.000000000000000000, -1.000000000000000000 ) ) ;
#31560=VERTEX_POINT ( 'NONE', #31831 ) ;
#31561=CIRCLE ( 'NONE', #73313, 0.06509327318403745899 ) ;
#31564=CONICAL_SURFACE ( 'NONE', #12757, 0.1000000000000000472, 0.003490658503988666988 ) ;
#31565=DIRECTION ( 'NONE',  ( 0.000000000000000000, 1.000000000000000000, 0.000000000000000000 ) ) ;
#31566=CARTESIAN_POINT ( 'NONE',  ( 0.4499999999999573785, 12.50000000000000000, -6.495190528383302464 ) ) ;
#31567=DIRECTION ( 'NONE',  ( 0.000000000000000000, 0.000000000000000000, -1.000000000000000000 ) ) ;
#31568=PLANE ( 'NONE',  #59865 ) ;
#31569=DIRECTION ( 'NONE',  ( -0.000000000000000000, 1.000000000000000000, -0.000000000000000000 ) ) ;
#31570=AXIS2_PLACEMENT_3D ( 'NONE', #88847, #8345, #70493 ) ;
#31571=EDGE_LOOP ( 'NONE', ( #63924, #114537 ) ) ;
#31572=ORIENTED_EDGE ( 'NONE', *, *, #31382, .T. ) ;
#31573=DIRECTION ( 'NONE',  ( -0.000000000000000000, 1.000000000000000000, -0.000000000000000000 ) ) ;
#31574=ORIENTED_EDGE ( 'NONE', *, *, #85901, .F. ) ;
#31575=AXIS2_PLACEMENT_3D ( 'NONE', #3547, #43488, #94489 ) ;
#31576=CARTESIAN_POINT ( 'NONE',  ( 0.8499999999999527933, 2.500000000000000000, 7.188010851410848723 ) ) ;
#31577=DIRECTION ( 'NONE',  ( 0.000000000000000000, 1.000000000000000000, 0.000000000000000000 ) ) ;
#31578=DIRECTION ( 'NONE',  ( -0.000000000000000000, -1.000000000000000000, -0.000000000000000000 ) ) ;
#31579=VERTEX_POINT ( 'NONE', #90085 ) ;
#31580=ORIENTED_EDGE ( 'NONE', *, *, #58085, .T. ) ;
#31581=FACE_BOUND ( 'NONE', #13063, .T. ) ;
#31582=EDGE_LOOP ( 'NONE', ( #82623, #79529, #90808, #86792 ) ) ;
#31583=EDGE_CURVE ( 'NONE', #56340, #79920, #50827, .T. ) ;
#31584=CARTESIAN_POINT ( 'NONE',  ( -2.700000000000031264, 2.500000000000000000, 4.776537180435972196 ) ) ;
#31585=LINE ( 'NONE', #58481, #106537 ) ;
#31586=EDGE_CURVE ( 'NONE', #115443, #91335, #120166, .T. ) ;
#31587=CARTESIAN_POINT ( 'NONE',  ( -9.600000000000008527, 2.500000000000000000, -4.330127018922197202 ) ) ;
#31588=FACE_OUTER_BOUND ( 'NONE', #1398, .T. ) ;
#31589=CARTESIAN_POINT ( 'NONE',  ( -4.600000000000028066, 2.500000000000000000, -3.637306695894650055 ) ) ;
#31590=EDGE_CURVE ( 'NONE', #77313, #25933, #53275, .T. ) ;
#31591=CARTESIAN_POINT ( 'NONE',  ( 13.09999999999989839, 2.500000000000000000, 0.2464101615137735679 ) ) ;
#31592=FACE_OUTER_BOUND ( 'NONE', #46084, .T. ) ;
#31593=DIRECTION ( 'NONE',  ( 0.000000000000000000, 1.000000000000000000, 0.000000000000000000 ) ) ;
#31594=DIRECTION ( 'NONE',  ( 0.000000000000000000, 0.000000000000000000, 1.000000000000000000 ) ) ;
#31595=DIRECTION ( 'NONE',  ( -0.000000000000000000, 1.000000000000000000, -0.000000000000000000 ) ) ;
#31597=ADVANCED_FACE ( 'NONE', ( #110382 ), #99933, .T. ) ;
#31599=ORIENTED_EDGE ( 'NONE', *, *, #124315, .T. ) ;
#31600=ORIENTED_EDGE ( 'NONE', *, *, #112844, .T. ) ;
#31601=EDGE_LOOP ( 'NONE', ( #28398, #125844, #61209, #82885 ) ) ;
#31602=FACE_OUTER_BOUND ( 'NONE', #73464, .T. ) ;
#31603=AXIS2_PLACEMENT_3D ( 'NONE', #1994, #32133, #123686 ) ;
#31604=FACE_OUTER_BOUND ( 'NONE', #67351, .T. ) ;
#31605=AXIS2_PLACEMENT_3D ( 'NONE', #19742, #97643, #129064 ) ;
#31606=AXIS2_PLACEMENT_3D ( 'NONE', #121944, #22477, #89896 ) ;
#31607=ORIENTED_EDGE ( 'NONE', *, *, #118265, .F. ) ;
#31608=EDGE_LOOP ( 'NONE', ( #97237, #42198, #119024, #80519 ) ) ;
#31609=VERTEX_POINT ( 'NONE', #1712 ) ;
#31610=CARTESIAN_POINT ( 'NONE',  ( 13.74999999999989519, 12.50000000000000000, -2.857883832488653741 ) ) ;
#31611=AXIS2_PLACEMENT_3D ( 'NONE', #106051, #56924, #107336 ) ;
#31612=CARTESIAN_POINT ( 'NONE',  ( -0.4500000000000397571, 2.500000000000000000, -2.065063509461102065 ) ) ;
#31613=CARTESIAN_POINT ( 'NONE',  ( -7.900000000000011013, 12.50000000000000000, 5.022947341949748790 ) ) ;
#31614=CARTESIAN_POINT ( 'NONE',  ( 9.599999999999914380, 2.500000000000000000, 5.022947341949748790 ) ) ;
#31615=DIRECTION ( 'NONE',  ( 0.000000000000000000, 0.000000000000000000, 1.000000000000000000 ) ) ;
#31616=CARTESIAN_POINT ( 'NONE',  ( 0.8499999999999545697, 2.500000000000000000, 2.957883832488649389 ) ) ;
#31617=AXIS2_PLACEMENT_3D ( 'NONE', #91830, #110185, #2150 ) ;
#31618=DIRECTION ( 'NONE',  ( -0.000000000000000000, -1.000000000000000000, -0.000000000000000000 ) ) ;
#31619=ADVANCED_FACE ( 'NONE', ( #29895 ), #69157, .T. ) ;
#31621=FACE_OUTER_BOUND ( 'NONE', #13332, .T. ) ;
#31622=ORIENTED_EDGE ( 'NONE', *, *, #112362, .F. ) ;
#31623=ORIENTED_EDGE ( 'NONE', *, *, #29341, .T. ) ;
#31624=ORIENTED_EDGE ( 'NONE', *, *, #127886, .F. ) ;
#31626=EDGE_LOOP ( 'NONE', ( #99723, #43494 ) ) ;
#31627=VERTEX_POINT ( 'NONE', #128768 ) ;
#31628=ORIENTED_EDGE ( 'NONE', *, *, #51957, .F. ) ;
#31629=DIRECTION ( 'NONE',  ( 0.000000000000000000, 1.000000000000000000, 0.000000000000000000 ) ) ;
#31630=AXIS2_PLACEMENT_3D ( 'NONE', #94861, #13707, #14976 ) ;
#31631=LINE ( 'NONE', #10667, #18346 ) ;
#31632=DIRECTION ( 'NONE',  ( 0.000000000000000000, 0.000000000000000000, -1.000000000000000000 ) ) ;
#31633=ADVANCED_FACE ( 'NONE', ( #111005 ), #50199, .T. ) ;
#31634=DIRECTION ( 'NONE',  ( 0.000000000000000000, 0.000000000000000000, 1.000000000000000000 ) ) ;
#31635=DIRECTION ( 'NONE',  ( 0.000000000000000000, -0.9999939076577903929, 0.003490651415223739937 ) ) ;
#31636=CARTESIAN_POINT ( 'NONE',  ( 3.549999999999942979, 2.500000000000000000, 1.718653347947321386 ) ) ;
#31637=CARTESIAN_POINT ( 'NONE',  ( 14.79999999999989235, 2.500000000000000000, 0.3464101615137735735 ) ) ;
#31638=CONICAL_SURFACE ( 'NONE', #48355, 0.1000000000000002554, 0.003490658503988666988 ) ;
#31639=EDGE_LOOP ( 'NONE', ( #49678, #3274 ) ) ;
#31640=DIRECTION ( 'NONE',  ( -0.000000000000000000, -1.000000000000000000, -0.000000000000000000 ) ) ;
#31641=VERTEX_POINT ( 'NONE', #20083 ) ;
#31642=DIRECTION ( 'NONE',  ( 0.000000000000000000, -0.9999939076577903929, 0.003490651415223739937 ) ) ;
#31643=EDGE_LOOP ( 'NONE', ( #40645, #122161 ) ) ;
#31644=DIRECTION ( 'NONE',  ( 0.000000000000000000, -0.9999939076577903929, 0.003490651415223739937 ) ) ;
#31645=EDGE_CURVE ( 'NONE', #8661, #1776, #113914, .T. ) ;
#31646=ORIENTED_EDGE ( 'NONE', *, *, #3032, .F. ) ;
#31648=CIRCLE ( 'NONE', #54610, 0.06509327318403745899 ) ;
#31649=DIRECTION ( 'NONE',  ( 0.000000000000000000, 0.000000000000000000, 1.000000000000000000 ) ) ;
#31650=ORIENTED_EDGE ( 'NONE', *, *, #4306, .F. ) ;
#31651=EDGE_LOOP ( 'NONE', ( #120345, #109295, #80158, #77559 ) ) ;
#31653=CARTESIAN_POINT ( 'NONE',  ( 8.749999999999920064, 12.50000000000000000, 5.802370205355744659 ) ) ;
#31655=DIRECTION ( 'NONE',  ( -4.274815082592931898E-19, -0.9999939076577903929, -0.003490651415223739937 ) ) ;
#31656=AXIS2_PLACEMENT_3D ( 'NONE', #118283, #37795, #128780 ) ;
#31657=CIRCLE ( 'NONE', #42122, 0.06509327318403745899 ) ;
#31658=DIRECTION ( 'NONE',  ( 0.000000000000000000, 1.000000000000000000, 0.000000000000000000 ) ) ;
#31659=ORIENTED_EDGE ( 'NONE', *, *, #40558, .T. ) ;
#31660=LINE ( 'NONE', #31043, #123995 ) ;
#31661=VECTOR ( 'NONE', #43601, 1000.000000000000000 ) ;
#31662=VECTOR ( 'NONE', #16059, 1000.000000000000000 ) ;
#31663=ORIENTED_EDGE ( 'NONE', *, *, #68878, .F. ) ;
#31664=FACE_OUTER_BOUND ( 'NONE', #79595, .T. ) ;
#31665=CARTESIAN_POINT ( 'NONE',  ( -6.071532165918824830E-15, 2.500000000000000000, -4.230127018922201998 ) ) ;
#31666=EDGE_CURVE ( 'NONE', #58654, #73675, #9535, .T. ) ;
#31667=VECTOR ( 'NONE', #85326, 1000.000000000000000 ) ;
#31668=CIRCLE ( 'NONE', #255, 0.09999999999999982514 ) ;
#31670=DIRECTION ( 'NONE',  ( 0.000000000000000000, 0.000000000000000000, -1.000000000000000000 ) ) ;
#31671=DIRECTION ( 'NONE',  ( 0.000000000000000000, 0.000000000000000000, 1.000000000000000000 ) ) ;
#31672=DIRECTION ( 'NONE',  ( -0.000000000000000000, -1.000000000000000000, -0.000000000000000000 ) ) ;
#31673=DIRECTION ( 'NONE',  ( 0.000000000000000000, 0.000000000000000000, -1.000000000000000000 ) ) ;
#31674=EDGE_LOOP ( 'NONE', ( #58470, #28915, #92467, #30273 ) ) ;
#31675=EDGE_CURVE ( 'NONE', #17546, #69331, #111944, .T. ) ;
#31676=CARTESIAN_POINT ( 'NONE',  ( 11.24999999999990585, 2.500000000000000000, -5.802370205355749988 ) ) ;
#31677=CARTESIAN_POINT ( 'NONE',  ( 105.5000000000000142, -1.500000000000000222, -1.322875655532295136 ) ) ;
#31678=CARTESIAN_POINT ( 'NONE',  ( -3.150000000000029221, 12.50000000000000000, 2.576566944158910744 ) ) ;
#31679=ADVANCED_FACE ( 'NONE', ( #40374 ), #99435, .T. ) ;
#31680=EDGE_CURVE ( 'NONE', #43214, #115043, #55505, .T. ) ;
#31681=EDGE_CURVE ( 'NONE', #22692, #101260, #63826, .T. ) ;
#31682=EDGE_CURVE ( 'NONE', #20502, #27204, #39743, .T. ) ;
#31684=DIRECTION ( 'NONE',  ( -0.000000000000000000, 1.000000000000000000, -0.000000000000000000 ) ) ;
#31685=ORIENTED_EDGE ( 'NONE', *, *, #111008, .T. ) ;
#31686=ORIENTED_EDGE ( 'NONE', *, *, #24370, .T. ) ;
#31687=DIRECTION ( 'NONE',  ( 0.000000000000000000, 0.000000000000000000, 1.000000000000000000 ) ) ;
#31688=ADVANCED_FACE ( 'NONE', ( #124068 ), #28314, .T. ) ;
#31689=CONICAL_SURFACE ( 'NONE', #104824, 0.09999999999999982514, 0.003490658503988666988 ) ;
#31690=AXIS2_PLACEMENT_3D ( 'NONE', #53848, #93771, #95710 ) ;
#31691=EDGE_CURVE ( 'NONE', #117766, #111163, #11579, .T. ) ;
#31693=CARTESIAN_POINT ( 'NONE',  ( 17.88933034088538676, -0.4802206367769989992, -4.999988745082089459 ) ) ;
#31694=FACE_OUTER_BOUND ( 'NONE', #101584, .T. ) ;
#31695=EDGE_CURVE ( 'NONE', #69772, #124524, #83519, .T. ) ;
#31696=DIRECTION ( 'NONE',  ( 0.000000000000000000, 0.000000000000000000, -1.000000000000000000 ) ) ;
#31697=ORIENTED_EDGE ( 'NONE', *, *, #45022, .T. ) ;
#31698=ADVANCED_FACE ( 'NONE', ( #122159 ), #49256, .T. ) ;
#31699=VECTOR ( 'NONE', #93507, 1000.000000000000000 ) ;
#31700=PLANE ( 'NONE',  #2775 ) ;
#31702=LINE ( 'NONE', #61156, #37030 ) ;
#31703=AXIS2_PLACEMENT_3D ( 'NONE', #40956, #80862, #31130 ) ;
#31704=ADVANCED_FACE ( 'NONE', ( #54048 ), #70084, .T. ) ;
#31705=ORIENTED_EDGE ( 'NONE', *, *, #126602, .F. ) ;
#31706=AXIS2_PLACEMENT_3D ( 'NONE', #56652, #96580, #104481 ) ;
#31707=ORIENTED_EDGE ( 'NONE', *, *, #51166, .F. ) ;
#31708=ORIENTED_EDGE ( 'NONE', *, *, #113933, .F. ) ;
#31709=DIRECTION ( 'NONE',  ( 0.000000000000000000, 1.000000000000000000, 0.000000000000000000 ) ) ;
#31710=DIRECTION ( 'NONE',  ( 0.000000000000000000, 1.000000000000000000, 0.000000000000000000 ) ) ;
#31711=CARTESIAN_POINT ( 'NONE',  ( -2.700000000000031264, 12.50000000000000000, 4.676537180435972552 ) ) ;
#31712=FACE_BOUND ( 'NONE', #10688, .T. ) ;
#31713=EDGE_LOOP ( 'NONE', ( #125580, #63145 ) ) ;
#31714=CARTESIAN_POINT ( 'NONE',  ( -5.200000000000020606, 2.500000000000000000, -0.3464101615137782364 ) ) ;
#31715=DIRECTION ( 'NONE',  ( -0.000000000000000000, -1.000000000000000000, -0.000000000000000000 ) ) ;
#31716=VERTEX_POINT ( 'NONE', #93972 ) ;
#31717=CARTESIAN_POINT ( 'NONE',  ( 5.649999999999936406, 12.50000000000000000, -6.148780366869526226 ) ) ;
#31718=CARTESIAN_POINT ( 'NONE',  ( -11.24999999999996447, 2.500000000000000000, -6.395190528383298378 ) ) ;
#31719=DIRECTION ( 'NONE',  ( 0.000000000000000000, 1.000000000000000000, 0.000000000000000000 ) ) ;
#31720=CARTESIAN_POINT ( 'NONE',  ( -1.450000000000035483, 2.500000000000000000, 1.718653347947321386 ) ) ;
#31721=DIRECTION ( 'NONE',  ( 0.000000000000000000, 0.000000000000000000, 1.000000000000000000 ) ) ;
#31722=DIRECTION ( 'NONE',  ( 0.000000000000000000, 0.000000000000000000, 1.000000000000000000 ) ) ;
#31723=DIRECTION ( 'NONE',  ( 0.000000000000000000, -0.000000000000000000, 1.000000000000000000 ) ) ;
#31724=CIRCLE ( 'NONE', #127864, 0.06509327318403745899 ) ;
#31725=VECTOR ( 'NONE', #106182, 1000.000000000000000 ) ;
#31726=ORIENTED_EDGE ( 'NONE', *, *, #61807, .F. ) ;
#31727=ORIENTED_EDGE ( 'NONE', *, *, #13933, .F. ) ;
#31728=ORIENTED_EDGE ( 'NONE', *, *, #113582, .T. ) ;
#31729=ORIENTED_EDGE ( 'NONE', *, *, #95695, .F. ) ;
#31730=DIRECTION ( 'NONE',  ( 0.000000000000000000, -0.9999939076577903929, 0.003490651415223739937 ) ) ;
#31731=CARTESIAN_POINT ( 'NONE',  ( 1.249999999999988898, 12.50000000000000000, -6.430097255199264339 ) ) ;
#31732=ORIENTED_EDGE ( 'NONE', *, *, #82729, .T. ) ;
#31733=FACE_BOUND ( 'NONE', #89027, .T. ) ;
#31734=VECTOR ( 'NONE', #39283, 1000.000000000000000 ) ;
#31735=FACE_OUTER_BOUND ( 'NONE', #80687, .T. ) ;
#31736=DIRECTION ( 'NONE',  ( -0.000000000000000000, -1.000000000000000000, -0.000000000000000000 ) ) ;
#31737=CONICAL_SURFACE ( 'NONE', #4593, 0.1000000000000000056, 0.003490658503988666988 ) ;
#31738=ADVANCED_FACE ( 'NONE', ( #23947 ), #95219, .T. ) ;
#31739=CIRCLE ( 'NONE', #34082, 0.06509327318403745899 ) ;
#31740=DIRECTION ( 'NONE',  ( 0.000000000000000000, 1.000000000000000000, 0.000000000000000000 ) ) ;
#31741=CIRCLE ( 'NONE', #90495, 0.1000000000000002554 ) ;
#31743=DIRECTION ( 'NONE',  ( -4.274815082592931898E-19, -0.9999939076577903929, -0.003490651415223739937 ) ) ;
#31744=EDGE_CURVE ( 'NONE', #65177, #50078, #44885, .T. ) ;
#31745=DIRECTION ( 'NONE',  ( 0.000000000000000000, 0.000000000000000000, 1.000000000000000000 ) ) ;
#31746=DIRECTION ( 'NONE',  ( 0.000000000000000000, 0.000000000000000000, 1.000000000000000000 ) ) ;
#31747=CARTESIAN_POINT ( 'NONE',  ( -13.54999999999999005, 2.500000000000000000, 2.511473670974877503 ) ) ;
#31748=FACE_OUTER_BOUND ( 'NONE', #61658, .T. ) ;
#31749=DIRECTION ( 'NONE',  ( -0.000000000000000000, 1.000000000000000000, -0.000000000000000000 ) ) ;
#31750=EDGE_LOOP ( 'NONE', ( #27475, #79644, #39199, #34153 ) ) ;
#31751=EDGE_CURVE ( 'NONE', #56139, #77490, #63868, .T. ) ;
#31752=EDGE_LOOP ( 'NONE', ( #77279, #125395, #128894, #66555 ) ) ;
#31753=PLANE ( 'NONE',  #4846 ) ;
#31754=AXIS2_PLACEMENT_3D ( 'NONE', #114129, #33642, #123937 ) ;
#31755=EDGE_CURVE ( 'NONE', #17445, #116268, #122786, .T. ) ;
#31756=ORIENTED_EDGE ( 'NONE', *, *, #24040, .F. ) ;
#31757=VERTEX_POINT ( 'NONE', #4270 ) ;
#31758=VERTEX_POINT ( 'NONE', #92032 ) ;
#31759=AXIS2_PLACEMENT_3D ( 'NONE', #26413, #104939, #65668 ) ;
#31760=ORIENTED_EDGE ( 'NONE', *, *, #45751, .F. ) ;
#31761=AXIS2_PLACEMENT_3D ( 'NONE', #47253, #18420, #87150 ) ;
#31762=CIRCLE ( 'NONE', #98622, 0.09999999999999982514 ) ;
#31763=CARTESIAN_POINT ( 'NONE',  ( 5.649999999999934630, 2.500000000000000000, 6.048780366869521252 ) ) ;
#31764=EDGE_LOOP ( 'NONE', ( #85081, #42050 ) ) ;
#31765=VERTEX_POINT ( 'NONE', #92680 ) ;
#31766=CONICAL_SURFACE ( 'NONE', #60988, 0.09999999999999982514, 0.003490658503988666988 ) ;
#31767=CARTESIAN_POINT ( 'NONE',  ( 12.89999999999990266, 2.500000000000000000, 5.022947341949748790 ) ) ;
#31768=DIRECTION ( 'NONE',  ( 0.000000000000000000, 0.000000000000000000, -1.000000000000000000 ) ) ;
#31769=DIRECTION ( 'NONE',  ( 0.000000000000000000, 0.000000000000000000, 1.000000000000000000 ) ) ;
#31770=CARTESIAN_POINT ( 'NONE',  ( -13.29999999999999005, 12.50000000000000000, 1.843143693225357538E-15 ) ) ;
#31771=EDGE_LOOP ( 'NONE', ( #4580, #30050 ) ) ;
#31772=DIRECTION ( 'NONE',  ( -0.000000000000000000, -1.000000000000000000, -0.000000000000000000 ) ) ;
#31773=VERTEX_POINT ( 'NONE', #53409 ) ;
#31774=ORIENTED_EDGE ( 'NONE', *, *, #120752, .T. ) ;
#31775=LINE ( 'NONE', #120151, #122141 ) ;
#31776=DIRECTION ( 'NONE',  ( 0.000000000000000000, 0.000000000000000000, 1.000000000000000000 ) ) ;
#31777=DIRECTION ( 'NONE',  ( 0.000000000000000000, 0.000000000000000000, -1.000000000000000000 ) ) ;
#31778=VERTEX_POINT ( 'NONE', #103790 ) ;
#31779=ORIENTED_EDGE ( 'NONE', *, *, #111159, .F. ) ;
#31780=ADVANCED_FACE ( 'NONE', ( #2340 ), #72247, .T. ) ;
#31781=CARTESIAN_POINT ( 'NONE',  ( -2.300000000000033129, 2.500000000000000000, 3.983716857408420076 ) ) ;
#31782=CARTESIAN_POINT ( 'NONE',  ( 1.249999999999988898, 2.500000000000000000, -6.495190528383302464 ) ) ;
#31784=CIRCLE ( 'NONE', #119591, 0.09999999999999982514 ) ;
#31785=DIRECTION ( 'NONE',  ( 0.000000000000000000, 1.000000000000000000, 0.000000000000000000 ) ) ;
#31786=ORIENTED_EDGE ( 'NONE', *, *, #76780, .F. ) ;
#31787=CIRCLE ( 'NONE', #33926, 0.06509327318403745899 ) ;
#31788=AXIS2_PLACEMENT_3D ( 'NONE', #70752, #71372, #120499 ) ;
#31789=CARTESIAN_POINT ( 'NONE',  ( -9.350000000000008527, 12.50000000000000000, -6.841600689897072485 ) ) ;
#31791=CARTESIAN_POINT ( 'NONE',  ( 11.75764115802628140, -2.499999999999999556, 7.679135278744470661 ) ) ;
#31792=AXIS2_PLACEMENT_3D ( 'NONE', #23812, #104916, #45390 ) ;
#31793=AXIS2_PLACEMENT_3D ( 'NONE', #17634, #116479, #115841 ) ;
#31794=ORIENTED_EDGE ( 'NONE', *, *, #106127, .F. ) ;
#31795=CARTESIAN_POINT ( 'NONE',  ( 87.50000000000002842, 6.761363245278263712, -3.308765358479923258 ) ) ;
#31796=CIRCLE ( 'NONE', #33836, 0.06509327318403745899 ) ;
#31797=PLANE ( 'NONE',  #96487 ) ;
#31798=CARTESIAN_POINT ( 'NONE',  ( 10.84999999999990905, 2.500000000000000000, 2.165063509461097713 ) ) ;
#31799=ADVANCED_FACE ( 'NONE', ( #14102 ), #22069, .T. ) ;
#31800=AXIS2_PLACEMENT_3D ( 'NONE', #114736, #107504, #27016 ) ;
#31801=DIRECTION ( 'NONE',  ( 0.000000000000000000, -0.9999939076577903929, 0.003490651415223739937 ) ) ;
#31802=EDGE_CURVE ( 'NONE', #63751, #35293, #38807, .T. ) ;
#31803=FACE_OUTER_BOUND ( 'NONE', #66794, .T. ) ;
#31804=ORIENTED_EDGE ( 'NONE', *, *, #124857, .F. ) ;
#31805=CIRCLE ( 'NONE', #52621, 0.1000000000000002554 ) ;
#31806=DIRECTION ( 'NONE',  ( -0.000000000000000000, 1.000000000000000000, -0.000000000000000000 ) ) ;
#31807=DIRECTION ( 'NONE',  ( 0.000000000000000000, 0.000000000000000000, 1.000000000000000000 ) ) ;
#31808=ORIENTED_EDGE ( 'NONE', *, *, #96341, .T. ) ;
#31809=EDGE_LOOP ( 'NONE', ( #57435, #4095, #73094, #46312 ) ) ;
#31810=EDGE_CURVE ( 'NONE', #25500, #91178, #62590, .T. ) ;
#31811=ORIENTED_EDGE ( 'NONE', *, *, #54920, .T. ) ;
#31812=DIRECTION ( 'NONE',  ( -0.000000000000000000, 1.000000000000000000, -0.000000000000000000 ) ) ;
#31813=LINE ( 'NONE', #119526, #15777 ) ;
#31815=CARTESIAN_POINT ( 'NONE',  ( 5.649999999999936406, 2.500000000000000000, -6.841600689897077814 ) ) ;
#31816=FACE_OUTER_BOUND ( 'NONE', #72332, .T. ) ;
#31817=FACE_OUTER_BOUND ( 'NONE', #114357, .T. ) ;
#31818=DIRECTION ( 'NONE',  ( 0.000000000000000000, -0.9999939076577903929, 0.003490651415223739937 ) ) ;
#31819=AXIS2_PLACEMENT_3D ( 'NONE', #84127, #73663, #93324 ) ;
#31820=EDGE_LOOP ( 'NONE', ( #100579, #13042, #2642, #66995 ) ) ;
#31822=DIRECTION ( 'NONE',  ( -0.000000000000000000, 1.000000000000000000, -0.000000000000000000 ) ) ;
#31823=DIRECTION ( 'NONE',  ( -0.000000000000000000, -1.000000000000000000, -0.000000000000000000 ) ) ;
#31824=DIRECTION ( 'NONE',  ( 0.000000000000000000, 0.000000000000000000, 1.000000000000000000 ) ) ;
#31825=CIRCLE ( 'NONE', #10860, 0.06509327318403745899 ) ;
#31826=AXIS2_PLACEMENT_3D ( 'NONE', #119349, #49999, #51287 ) ;
#31827=ORIENTED_EDGE ( 'NONE', *, *, #80353, .T. ) ;
#31828=DIRECTION ( 'NONE',  ( 0.000000000000000000, 0.000000000000000000, 1.000000000000000000 ) ) ;
#31829=ADVANCED_FACE ( 'NONE', ( #12806 ), #93330, .T. ) ;
#31830=VECTOR ( 'NONE', #57913, 1000.000000000000000 ) ;
#31831=CARTESIAN_POINT ( 'NONE',  ( -9.350000000000004974, 2.500000000000000000, 6.741600689897071952 ) ) ;
#31832=DIRECTION ( 'NONE',  ( 0.000000000000000000, 1.000000000000000000, 0.000000000000000000 ) ) ;
#31833=ORIENTED_EDGE ( 'NONE', *, *, #49112, .F. ) ;
#31834=ADVANCED_FACE ( 'NONE', ( #73041 ), #32540, .T. ) ;
#31835=EDGE_CURVE ( 'NONE', #88926, #17926, #16033, .T. ) ;
#31836=EDGE_CURVE ( 'NONE', #68676, #113589, #95268, .T. ) ;
#31837=ORIENTED_EDGE ( 'NONE', *, *, #98731, .F. ) ;
#31838=DIRECTION ( 'NONE',  ( -0.000000000000000000, 1.000000000000000000, -0.000000000000000000 ) ) ;
#31839=CIRCLE ( 'NONE', #44350, 0.06509327318403745899 ) ;
#31840=ORIENTED_EDGE ( 'NONE', *, *, #122973, .F. ) ;
#31841=CIRCLE ( 'NONE', #125911, 0.09999999999999982514 ) ;
#31842=CIRCLE ( 'NONE', #21466, 0.09999999999999982514 ) ;
#31843=ORIENTED_EDGE ( 'NONE', *, *, #99351, .F. ) ;
#31844=AXIS2_PLACEMENT_3D ( 'NONE', #127069, #36761, #64900 ) ;
#31845=PLANE ( 'NONE',  #80170 ) ;
#31846=ADVANCED_FACE ( 'NONE', ( #86725 ), #109889, .T. ) ;
#31847=ADVANCED_FACE ( 'NONE', ( #87992 ), #126616, .T. ) ;
#31848=EDGE_CURVE ( 'NONE', #126587, #116590, #103531, .T. ) ;
#31849=AXIS2_PLACEMENT_3D ( 'NONE', #83084, #93536, #81768 ) ;
#31850=CARTESIAN_POINT ( 'NONE',  ( -1.700000000000034817, 2.500000000000000000, 0.09999999999999761857 ) ) ;
#31851=CARTESIAN_POINT ( 'NONE',  ( -1.450000000000035483, 2.500000000000000000, 6.248780366869521430 ) ) ;
#31853=VERTEX_POINT ( 'NONE', #36359 ) ;
#31854=EDGE_CURVE ( 'NONE', #106131, #56932, #30394, .T. ) ;
#31855=FACE_OUTER_BOUND ( 'NONE', #109151, .T. ) ;
#31856=EDGE_LOOP ( 'NONE', ( #120952, #58498, #93108, #42968 ) ) ;
#31857=FACE_OUTER_BOUND ( 'NONE', #44225, .T. ) ;
#31858=EDGE_CURVE ( 'NONE', #108453, #97422, #97262, .T. ) ;
#31859=CARTESIAN_POINT ( 'NONE',  ( -5.850000000000021849, 2.500000000000000000, -2.857883832488653741 ) ) ;
#31860=EDGE_CURVE ( 'NONE', #63793, #90411, #57572, .T. ) ;
#31861=EDGE_LOOP ( 'NONE', ( #28954, #56606, #115798, #72902 ) ) ;
#31862=ORIENTED_EDGE ( 'NONE', *, *, #95922, .F. ) ;
#31863=ORIENTED_EDGE ( 'NONE', *, *, #99106, .F. ) ;
#31864=VERTEX_POINT ( 'NONE', #35700 ) ;
#31865=CARTESIAN_POINT ( 'NONE',  ( -4.800000000000022915, 12.50000000000000000, 3.983716857408420076 ) ) ;
#31866=CARTESIAN_POINT ( 'NONE',  ( 1.649999999999950617, 12.50000000000000000, -2.099970236277064473 ) ) ;
#31867=FACE_BOUND ( 'NONE', #46609, .T. ) ;
#31868=VERTEX_POINT ( 'NONE', #76907 ) ;
#31869=DIRECTION ( 'NONE',  ( 0.000000000000000000, -0.9999939076577903929, 0.003490651415223739937 ) ) ;
#31871=CARTESIAN_POINT ( 'NONE',  ( 0.000000000000000000, 2.500000000000000000, -8.999999999999998224 ) ) ;
#31872=CARTESIAN_POINT ( 'NONE',  ( 10.84999999999990905, 12.50000000000000000, 2.922977105672686982 ) ) ;
#31873=CONICAL_SURFACE ( 'NONE', #107159, 0.09999999999999982514, 0.003490658503988666988 ) ;
#31874=AXIS2_PLACEMENT_3D ( 'NONE', #80543, #120456, #58333 ) ;
#31875=CARTESIAN_POINT ( 'NONE',  ( 15.19999999999989271, 2.500000000000000000, -0.3464101615137783474 ) ) ;
#31876=CIRCLE ( 'NONE', #105014, 0.06509327318403745899 ) ;
#31877=DIRECTION ( 'NONE',  ( 0.000000000000000000, -0.000000000000000000, 1.000000000000000000 ) ) ;
#31878=CARTESIAN_POINT ( 'NONE',  ( -6.249999999999981348, 12.50000000000000000, 6.495190528383297135 ) ) ;
#31879=AXIS2_PLACEMENT_3D ( 'NONE', #73312, #73971, #113238 ) ;
#31880=DIRECTION ( 'NONE',  ( -4.274815082592931898E-19, -0.9999939076577903929, -0.003490651415223739937 ) ) ;
#31881=CONICAL_SURFACE ( 'NONE', #105022, 0.09999999999999982514, 0.003490658503988666988 ) ;
#31882=ORIENTED_EDGE ( 'NONE', *, *, #88997, .F. ) ;
#31883=VERTEX_POINT ( 'NONE', #127942 ) ;
#31885=EDGE_LOOP ( 'NONE', ( #70207, #58153 ) ) ;
#31886=VECTOR ( 'NONE', #84065, 1000.000000000000000 ) ;
#31887=EDGE_LOOP ( 'NONE', ( #66301, #72796, #78817, #72856 ) ) ;
#31889=CONICAL_SURFACE ( 'NONE', #88291, 0.1000000000000002554, 0.003490658503988666988 ) ;
#31890=CARTESIAN_POINT ( 'NONE',  ( -7.100000000000014744, 2.500000000000000000, 4.430127018922196847 ) ) ;
#31891=ORIENTED_EDGE ( 'NONE', *, *, #50023, .T. ) ;
#31892=FACE_BOUND ( 'NONE', #39959, .T. ) ;
#31893=CIRCLE ( 'NONE', #113356, 0.06509327318403745899 ) ;
#31894=FACE_OUTER_BOUND ( 'NONE', #1479, .T. ) ;
#31895=EDGE_CURVE ( 'NONE', #97989, #20397, #74291, .T. ) ;
#31896=EDGE_CURVE ( 'NONE', #83631, #87862, #112028, .T. ) ;
#31897=VERTEX_POINT ( 'NONE', #57924 ) ;
#31898=CARTESIAN_POINT ( 'NONE',  ( -6.650000000000018119, 2.500000000000000000, -7.288010851410854585 ) ) ;
#31899=DIRECTION ( 'NONE',  ( 0.000000000000000000, 0.000000000000000000, -1.000000000000000000 ) ) ;
#31900=DIRECTION ( 'NONE',  ( 0.000000000000000000, 1.000000000000000000, 0.000000000000000000 ) ) ;
#31901=DIRECTION ( 'NONE',  ( 0.000000000000000000, 0.000000000000000000, 1.000000000000000000 ) ) ;
#31902=EDGE_LOOP ( 'NONE', ( #76291, #84501, #33757, #71063 ) ) ;
#31903=FACE_OUTER_BOUND ( 'NONE', #12249, .T. ) ;
#31904=AXIS2_PLACEMENT_3D ( 'NONE', #21888, #12038, #51987 ) ;
#31905=VERTEX_POINT ( 'NONE', #75601 ) ;
#31906=ORIENTED_EDGE ( 'NONE', *, *, #87389, .F. ) ;
#31907=ORIENTED_EDGE ( 'NONE', *, *, #93575, .T. ) ;
#31908=DIRECTION ( 'NONE',  ( -0.000000000000000000, 1.000000000000000000, -0.000000000000000000 ) ) ;
#31909=CARTESIAN_POINT ( 'NONE',  ( -2.700000000000030820, 12.50000000000000000, -3.983716857408426293 ) ) ;
#31910=EDGE_LOOP ( 'NONE', ( #51352, #41870, #4303, #26707 ) ) ;
#31911=CARTESIAN_POINT ( 'NONE',  ( -6.450000000000014388, 12.50000000000000000, 6.083687093685483660 ) ) ;
#31912=CONICAL_SURFACE ( 'NONE', #65336, 0.1000000000000000472, 0.003490658503988666988 ) ;
#31913=AXIS2_PLACEMENT_3D ( 'NONE', #44185, #74306, #95236 ) ;
#31914=DIRECTION ( 'NONE',  ( 0.000000000000000000, 1.000000000000000000, 0.000000000000000000 ) ) ;
#31915=PLANE ( 'NONE',  #39455 ) ;
#31916=FACE_OUTER_BOUND ( 'NONE', #10286, .T. ) ;
#31918=EDGE_LOOP ( 'NONE', ( #111154, #119249, #49947, #58642 ) ) ;
#31919=CARTESIAN_POINT ( 'NONE',  ( 3.949999999999940670, 12.50000000000000000, 1.818653347947321475 ) ) ;
#31920=AXIS2_PLACEMENT_3D ( 'NONE', #108314, #77560, #49419 ) ;
#31921=ORIENTED_EDGE ( 'NONE', *, *, #123415, .F. ) ;
#31922=CARTESIAN_POINT ( 'NONE',  ( 1.899999999999949507, 12.50000000000000000, 4.676537180435972552 ) ) ;
#31923=VECTOR ( 'NONE', #103596, 1000.000000000000000 ) ;
#31924=CIRCLE ( 'NONE', #10955, 0.09999999999999982514 ) ;
#31925=EDGE_LOOP ( 'NONE', ( #88584, #99379, #103054, #125136 ) ) ;
#31927=CARTESIAN_POINT ( 'NONE',  ( 1.649999999999951505, 2.500000000000000000, 2.857883832488649301 ) ) ;
#31928=VERTEX_POINT ( 'NONE', #97193 ) ;
#31929=DIRECTION ( 'NONE',  ( -4.274815082592931898E-19, -0.9999939076577903929, -0.003490651415223739937 ) ) ;
#31930=DIRECTION ( 'NONE',  ( -0.000000000000000000, -1.000000000000000000, -0.000000000000000000 ) ) ;
#31931=CARTESIAN_POINT ( 'NONE',  ( -10.40000000000000391, 12.50000000000000000, -3.637306695894645614 ) ) ;
#31932=DIRECTION ( 'NONE',  ( 0.000000000000000000, 1.000000000000000000, 0.000000000000000000 ) ) ;
#31933=DIRECTION ( 'NONE',  ( 0.000000000000000000, 0.000000000000000000, 1.000000000000000000 ) ) ;
#31934=AXIS2_PLACEMENT_3D ( 'NONE', #28807, #8490, #99484 ) ;
#31935=VERTEX_POINT ( 'NONE', #115519 ) ;
#31936=ORIENTED_EDGE ( 'NONE', *, *, #80339, .F. ) ;
#31937=CIRCLE ( 'NONE', #84138, 0.06509327318403741736 ) ;
#31938=EDGE_CURVE ( 'NONE', #28339, #116464, #105728, .T. ) ;
#31939=EDGE_LOOP ( 'NONE', ( #36615, #39684, #126377, #121351 ) ) ;
#31940=CARTESIAN_POINT ( 'NONE',  ( 11.64999999999990443, 12.50000000000000000, 1.407149913249508000 ) ) ;
#31941=CARTESIAN_POINT ( 'NONE',  ( -10.85000000000000142, 2.500000000000000000, -5.702370205355745902 ) ) ;
#31942=VECTOR ( 'NONE', #24865, 1000.000000000000000 ) ;
#31943=VECTOR ( 'NONE', #68124, 1000.000000000000000 ) ;
#31944=CARTESIAN_POINT ( 'NONE',  ( 9.549999999999918998, 12.50000000000000000, 2.165063509461097713 ) ) ;
#31945=EDGE_LOOP ( 'NONE', ( #27379, #8814, #30290, #34994 ) ) ;
#31946=ORIENTED_EDGE ( 'NONE', *, *, #14435, .T. ) ;
#31947=VERTEX_POINT ( 'NONE', #46151 ) ;
#31949=VECTOR ( 'NONE', #118326, 1000.000000000000000 ) ;
#31950=EDGE_LOOP ( 'NONE', ( #2429, #104518, #128921, #94351 ) ) ;
#31951=FACE_OUTER_BOUND ( 'NONE', #10259, .T. ) ;
#31952=ADVANCED_FACE ( 'NONE', ( #116821 ), #61869, .T. ) ;
#31953=FACE_OUTER_BOUND ( 'NONE', #50549, .T. ) ;
#31954=DIRECTION ( 'NONE',  ( 0.000000000000000000, 1.000000000000000000, 0.000000000000000000 ) ) ;
#31955=AXIS2_PLACEMENT_3D ( 'NONE', #97412, #28688, #59456 ) ;
#31956=DIRECTION ( 'NONE',  ( -0.000000000000000000, -1.000000000000000000, -0.000000000000000000 ) ) ;
#31957=DIRECTION ( 'NONE',  ( 0.000000000000000000, 0.000000000000000000, 1.000000000000000000 ) ) ;
#31958=DIRECTION ( 'NONE',  ( -4.274815082592931898E-19, -0.9999939076577903929, -0.003490651415223739937 ) ) ;
#31959=DIRECTION ( 'NONE',  ( 0.000000000000000000, -0.000000000000000000, 1.000000000000000000 ) ) ;
#31960=EDGE_CURVE ( 'NONE', #74521, #34772, #22172, .T. ) ;
#31961=ADVANCED_FACE ( 'NONE', ( #6847 ), #13717, .T. ) ;
#31962=DIRECTION ( 'NONE',  ( 0.000000000000000000, 0.000000000000000000, 1.000000000000000000 ) ) ;
#31963=EDGE_LOOP ( 'NONE', ( #125188, #58814, #58710, #107341 ) ) ;
#31964=CARTESIAN_POINT ( 'NONE',  ( -5.650000000000023448, 2.500000000000000000, -2.511473670974877948 ) ) ;
#31965=ADVANCED_FACE ( 'NONE', ( #77540 ), #80642, .T. ) ;
#31966=CARTESIAN_POINT ( 'NONE',  ( 76.45351065593905560, -3.568406926272937874, 6.085611128998389852 ) ) ;
#31967=ORIENTED_EDGE ( 'NONE', *, *, #71849, .F. ) ;
#31968=EDGE_LOOP ( 'NONE', ( #60226, #37645, #37676, #16483 ) ) ;
#31969=AXIS2_PLACEMENT_3D ( 'NONE', #48521, #129040, #53 ) ;
#31970=CIRCLE ( 'NONE', #105093, 0.06509327318403745899 ) ;
#31971=ADVANCED_FACE ( 'NONE', ( #8155 ), #70172, .T. ) ;
#31973=CARTESIAN_POINT ( 'NONE',  ( 5.849999999999932143, 12.50000000000000000, 1.472243186433545459 ) ) ;
#31974=CARTESIAN_POINT ( 'NONE',  ( 8.349999999999919709, 2.500000000000000000, -1.472243186433550122 ) ) ;
#31975=CARTESIAN_POINT ( 'NONE',  ( -1.250000000000001554, 2.500000000000000000, 6.595190528383296780 ) ) ;
#31976=DIRECTION ( 'NONE',  ( 0.000000000000000000, 0.000000000000000000, 1.000000000000000000 ) ) ;
#31977=DIRECTION ( 'NONE',  ( 0.000000000000000000, 0.000000000000000000, 1.000000000000000000 ) ) ;
#31978=CONICAL_SURFACE ( 'NONE', #17358, 0.1000000000000002554, 0.003490658503988666988 ) ;
#31979=CARTESIAN_POINT ( 'NONE',  ( 8.149999999999923972, 2.500000000000000000, -6.148780366869526226 ) ) ;
#31980=CARTESIAN_POINT ( 'NONE',  ( 4.399999999999937295, 12.50000000000000000, 3.918623584224383727 ) ) ;
#31981=CONICAL_SURFACE ( 'NONE', #98758, 0.09999999999999982514, 0.003490658503988666988 ) ;
#31982=AXIS2_PLACEMENT_3D ( 'NONE', #35670, #74308, #44853 ) ;
#31983=DIRECTION ( 'NONE',  ( 0.000000000000000000, 0.000000000000000000, 1.000000000000000000 ) ) ;
#31984=VERTEX_POINT ( 'NONE', #50669 ) ;
#31985=AXIS2_PLACEMENT_3D ( 'NONE', #60340, #9929, #38109 ) ;
#31986=ORIENTED_EDGE ( 'NONE', *, *, #48014, .F. ) ;
#31987=CIRCLE ( 'NONE', #48706, 0.06509327318403745899 ) ;
#31988=CONICAL_SURFACE ( 'NONE', #6802, 0.1000000000000002554, 0.003490658503988666988 ) ;
#31989=ORIENTED_EDGE ( 'NONE', *, *, #56500, .F. ) ;
#31990=AXIS2_PLACEMENT_3D ( 'NONE', #90505, #81356, #847 ) ;
#31991=AXIS2_PLACEMENT_3D ( 'NONE', #101095, #20611, #31092 ) ;
#31992=ORIENTED_EDGE ( 'NONE', *, *, #122307, .T. ) ;
#31993=FACE_OUTER_BOUND ( 'NONE', #12049, .T. ) ;
#31994=FACE_OUTER_BOUND ( 'NONE', #85985, .T. ) ;
#31995=AXIS2_PLACEMENT_3D ( 'NONE', #30543, #72395, #23259 ) ;
#31996=ORIENTED_EDGE ( 'NONE', *, *, #54442, .F. ) ;
#31997=FACE_OUTER_BOUND ( 'NONE', #26607, .T. ) ;
#31998=ADVANCED_FACE ( 'NONE', ( #50056 ), #24204, .T. ) ;
#31999=DIRECTION ( 'NONE',  ( 0.000000000000000000, -0.9999939076577903929, 0.003490651415223739937 ) ) ;
#32000=FACE_OUTER_BOUND ( 'NONE', #109169, .T. ) ;
#32001=DIRECTION ( 'NONE',  ( 0.000000000000000000, 1.000000000000000000, 0.000000000000000000 ) ) ;
#32002=VERTEX_POINT ( 'NONE', #40880 ) ;
#32003=ADVANCED_FACE ( 'NONE', ( #39597 ), #91093, .T. ) ;
#32004=DIRECTION ( 'NONE',  ( 0.000000000000000000, 1.000000000000000000, 0.000000000000000000 ) ) ;
#32005=ADVANCED_FACE ( 'NONE', ( #120059 ), #47190, .T. ) ;
#32006=AXIS2_PLACEMENT_3D ( 'NONE', #41536, #60528, #81443 ) ;
#32007=CARTESIAN_POINT ( 'NONE',  ( 8.099999999999923261, 2.500000000000000000, -3.983716857408426293 ) ) ;
#32008=ORIENTED_EDGE ( 'NONE', *, *, #75595, .T. ) ;
#32009=ORIENTED_EDGE ( 'NONE', *, *, #68733, .T. ) ;
#32010=VERTEX_POINT ( 'NONE', #1561 ) ;
#32011=VERTEX_POINT ( 'NONE', #30413 ) ;
#32012=DIRECTION ( 'NONE',  ( -0.000000000000000000, 1.000000000000000000, -0.000000000000000000 ) ) ;
#32013=EDGE_CURVE ( 'NONE', #6668, #36299, #82802, .T. ) ;
#32014=ADVANCED_FACE ( 'NONE', ( #31057 ), #30485, .T. ) ;
#32015=EDGE_CURVE ( 'NONE', #56105, #85940, #95304, .T. ) ;
#32016=EDGE_CURVE ( 'NONE', #10801, #5618, #108925, .T. ) ;
#32017=LINE ( 'NONE', #12346, #90571 ) ;
#32018=AXIS2_PLACEMENT_3D ( 'NONE', #66911, #106833, #119091 ) ;
#32019=DIRECTION ( 'NONE',  ( -0.000000000000000000, -1.000000000000000000, -0.000000000000000000 ) ) ;
#32020=AXIS2_PLACEMENT_3D ( 'NONE', #123317, #104944, #56499 ) ;
#32021=ORIENTED_EDGE ( 'NONE', *, *, #63, .F. ) ;
#32022=EDGE_CURVE ( 'NONE', #78167, #5697, #101563, .T. ) ;
#32023=LINE ( 'NONE', #100725, #46043 ) ;
#32024=EDGE_LOOP ( 'NONE', ( #123851, #82598, #67197, #27906 ) ) ;
#32025=LINE ( 'NONE', #92202, #72600 ) ;
#32026=CARTESIAN_POINT ( 'NONE',  ( 16.55874544816221317, -0.4845305829210151960, -6.091953208799018249 ) ) ;
#32027=DIRECTION ( 'NONE',  ( -0.000000000000000000, -1.000000000000000000, -0.000000000000000000 ) ) ;
#32028=CARTESIAN_POINT ( 'NONE',  ( 5.849999999999933920, 2.500000000000000000, 5.902370205355745192 ) ) ;
#32029=CIRCLE ( 'NONE', #4793, 0.06509327318403745899 ) ;
#32031=EDGE_CURVE ( 'NONE', #90584, #47691, #15871, .T. ) ;
#32032=VECTOR ( 'NONE', #128365, 1000.000000000000000 ) ;
#32033=VERTEX_POINT ( 'NONE', #118763 ) ;
#32034=CONICAL_SURFACE ( 'NONE', #84226, 0.1000000000000002554, 0.003490658503988666988 ) ;
#32035=ORIENTED_EDGE ( 'NONE', *, *, #13621, .F. ) ;
#32036=ORIENTED_EDGE ( 'NONE', *, *, #85429, .T. ) ;
#32037=CARTESIAN_POINT ( 'NONE',  ( 4.999999999999938716, 2.500000000000000000, -4.922947341949753586 ) ) ;
#32038=DIRECTION ( 'NONE',  ( -0.000000000000000000, 1.000000000000000000, -0.000000000000000000 ) ) ;
#32039=CARTESIAN_POINT ( 'NONE',  ( 1.249999999999952038, 12.50000000000000000, 5.802370205355744659 ) ) ;
#32040=FACE_BOUND ( 'NONE', #93401, .T. ) ;
#32041=CARTESIAN_POINT ( 'NONE',  ( 10.59999999999991260, 2.500000000000000000, 0.3464101615137735735 ) ) ;
#32042=AXIS2_PLACEMENT_3D ( 'NONE', #55535, #35888, #75796 ) ;
#32043=DIRECTION ( 'NONE',  ( 0.000000000000000000, -0.000000000000000000, 1.000000000000000000 ) ) ;
#32044=FACE_OUTER_BOUND ( 'NONE', #19473, .T. ) ;
#32045=CONICAL_SURFACE ( 'NONE', #80051, 0.09999999999999982514, 0.003490658503988666988 ) ;
#32046=CIRCLE ( 'NONE', #69669, 0.06509327318403745899 ) ;
#32048=DIRECTION ( 'NONE',  ( 0.000000000000000000, -0.9999939076577903929, 0.003490651415223739937 ) ) ;
#32049=DIRECTION ( 'NONE',  ( 0.000000000000000000, 0.000000000000000000, -1.000000000000000000 ) ) ;
#32050=DIRECTION ( 'NONE',  ( 0.000000000000000000, 0.000000000000000000, -1.000000000000000000 ) ) ;
#32051=EDGE_LOOP ( 'NONE', ( #37068, #122020 ) ) ;
#32052=DIRECTION ( 'NONE',  ( -0.000000000000000000, -1.000000000000000000, -0.000000000000000000 ) ) ;
#32053=CARTESIAN_POINT ( 'NONE',  ( 6.649999999999931966, 12.50000000000000000, -7.188010851410854052 ) ) ;
#32054=AXIS2_PLACEMENT_3D ( 'NONE', #76343, #48825, #86793 ) ;
#32055=EDGE_LOOP ( 'NONE', ( #4427, #125352 ) ) ;
#32056=ORIENTED_EDGE ( 'NONE', *, *, #119322, .T. ) ;
#32057=CARTESIAN_POINT ( 'NONE',  ( 7.099999999999927702, 2.500000000000000000, 5.022947341949748790 ) ) ;
#32058=DIRECTION ( 'NONE',  ( 0.000000000000000000, 0.000000000000000000, 1.000000000000000000 ) ) ;
#32059=FACE_BOUND ( 'NONE', #9868, .T. ) ;
#32060=LINE ( 'NONE', #43812, #124591 ) ;
#32061=ADVANCED_FACE ( 'NONE', ( #8796 ), #107819, .T. ) ;
#32062=CIRCLE ( 'NONE', #59253, 0.06509327318403745899 ) ;
#32063=ORIENTED_EDGE ( 'NONE', *, *, #33319, .F. ) ;
#32064=DIRECTION ( 'NONE',  ( 0.000000000000000000, 0.000000000000000000, 1.000000000000000000 ) ) ;
#32065=AXIS2_PLACEMENT_3D ( 'NONE', #118846, #48836, #98541 ) ;
#32067=EDGE_LOOP ( 'NONE', ( #82801, #126818 ) ) ;
#32068=DIRECTION ( 'NONE',  ( 0.000000000000000000, 0.000000000000000000, 1.000000000000000000 ) ) ;
#32069=FACE_OUTER_BOUND ( 'NONE', #69876, .T. ) ;
#32070=EDGE_CURVE ( 'NONE', #49864, #179, #57653, .T. ) ;
#32071=AXIS2_PLACEMENT_3D ( 'NONE', #47461, #69020, #46824 ) ;
#32072=CONICAL_SURFACE ( 'NONE', #40383, 0.1000000000000002554, 0.003490658503988666988 ) ;
#32073=AXIS2_PLACEMENT_3D ( 'NONE', #101031, #60485, #42785 ) ;
#32074=ORIENTED_EDGE ( 'NONE', *, *, #104631, .F. ) ;
#32075=DIRECTION ( 'NONE',  ( -0.000000000000000000, 1.000000000000000000, -0.000000000000000000 ) ) ;
#32076=DIRECTION ( 'NONE',  ( 0.000000000000000000, 1.000000000000000000, 0.000000000000000000 ) ) ;
#32077=CIRCLE ( 'NONE', #38333, 0.06509327318403745899 ) ;
#32078=AXIS2_PLACEMENT_3D ( 'NONE', #11534, #51477, #31828 ) ;
#32079=ORIENTED_EDGE ( 'NONE', *, *, #69792, .T. ) ;
#32080=DIRECTION ( 'NONE',  ( 0.000000000000000000, 0.000000000000000000, 1.000000000000000000 ) ) ;
#32081=DIRECTION ( 'NONE',  ( 0.000000000000000000, 0.000000000000000000, -1.000000000000000000 ) ) ;
#32082=DIRECTION ( 'NONE',  ( -0.000000000000000000, -1.000000000000000000, 0.000000000000000000 ) ) ;
#32083=CIRCLE ( 'NONE', #90554, 0.06509327318403745899 ) ;
#32084=EDGE_LOOP ( 'NONE', ( #127991, #95354 ) ) ;
#32085=ORIENTED_EDGE ( 'NONE', *, *, #122403, .T. ) ;
#32086=DIRECTION ( 'NONE',  ( 0.000000000000000000, 1.000000000000000000, 0.000000000000000000 ) ) ;
#32087=AXIS2_PLACEMENT_3D ( 'NONE', #60328, #1370, #9914 ) ;
#32088=VERTEX_POINT ( 'NONE', #9461 ) ;
#32089=LINE ( 'NONE', #62824, #72136 ) ;
#32091=DIRECTION ( 'NONE',  ( -0.000000000000000000, 1.000000000000000000, -0.000000000000000000 ) ) ;
#32092=ORIENTED_EDGE ( 'NONE', *, *, #80299, .T. ) ;
#32093=CARTESIAN_POINT ( 'NONE',  ( -5.650000000000023448, 12.50000000000000000, -6.213873640053564351 ) ) ;
#32094=CARTESIAN_POINT ( 'NONE',  ( 7.949999999999925571, 2.500000000000000000, 2.065063509461097624 ) ) ;
#32095=DIRECTION ( 'NONE',  ( 0.000000000000000000, 1.000000000000000000, 0.000000000000000000 ) ) ;
#32096=FACE_OUTER_BOUND ( 'NONE', #54216, .T. ) ;
#32097=CARTESIAN_POINT ( 'NONE',  ( 1.249999999999954259, 2.500000000000000000, -7.188010851410854052 ) ) ;
#32098=CARTESIAN_POINT ( 'NONE',  ( 4.599999999999940137, 12.50000000000000000, -4.330127018922201643 ) ) ;
#32099=CIRCLE ( 'NONE', #105233, 0.09999999999999999167 ) ;
#32100=ORIENTED_EDGE ( 'NONE', *, *, #128348, .T. ) ;
#32101=ORIENTED_EDGE ( 'NONE', *, *, #7076, .F. ) ;
#32103=ORIENTED_EDGE ( 'NONE', *, *, #119597, .T. ) ;
#32104=CARTESIAN_POINT ( 'NONE',  ( 3.149999999999946176, 2.500000000000000000, -6.048780366869526581 ) ) ;
#32105=ORIENTED_EDGE ( 'NONE', *, *, #37618, .T. ) ;
#32106=ORIENTED_EDGE ( 'NONE', *, *, #33064, .T. ) ;
#32107=ORIENTED_EDGE ( 'NONE', *, *, #86638, .T. ) ;
#32108=DIRECTION ( 'NONE',  ( -0.000000000000000000, 1.000000000000000000, -0.000000000000000000 ) ) ;
#32109=VECTOR ( 'NONE', #104594, 1000.000000000000000 ) ;
#32110=CIRCLE ( 'NONE', #67676, 0.1000000000000002554 ) ;
#32111=DIRECTION ( 'NONE',  ( 0.000000000000000000, 0.000000000000000000, 1.000000000000000000 ) ) ;
#32112=EDGE_CURVE ( 'NONE', #102565, #125530, #1213, .T. ) ;
#32113=AXIS2_PLACEMENT_3D ( 'NONE', #110404, #11554, #120239 ) ;
#32114=CARTESIAN_POINT ( 'NONE',  ( -12.09999999999999609, 2.500000000000000000, -3.637306695894647390 ) ) ;
#32115=CARTESIAN_POINT ( 'NONE',  ( -2.700000000000030820, 12.50000000000000000, -4.048810130592463530 ) ) ;
#32116=FACE_OUTER_BOUND ( 'NONE', #104746, .T. ) ;
#32117=DIRECTION ( 'NONE',  ( -4.274815082592931898E-19, -0.9999939076577903929, -0.003490651415223739937 ) ) ;
#32118=DIRECTION ( 'NONE',  ( 0.000000000000000000, -0.9999939076577903929, 0.003490651415223739937 ) ) ;
#32119=FACE_OUTER_BOUND ( 'NONE', #17270, .T. ) ;
#32120=ADVANCED_FACE ( 'NONE', ( #58570 ), #99778, .T. ) ;
#32121=AXIS2_PLACEMENT_3D ( 'NONE', #28816, #9164, #68719 ) ;
#32122=EDGE_CURVE ( 'NONE', #87037, #16575, #118279, .T. ) ;
#32123=CIRCLE ( 'NONE', #27895, 0.1000000000000002554 ) ;
#32126=EDGE_LOOP ( 'NONE', ( #68539, #116980, #16479, #99340 ) ) ;
#32127=AXIS2_PLACEMENT_3D ( 'NONE', #42642, #82556, #11855 ) ;
#32128=EDGE_CURVE ( 'NONE', #45762, #120531, #59225, .T. ) ;
#32129=DIRECTION ( 'NONE',  ( -4.274815082592931898E-19, -0.9999939076577903929, -0.003490651415223739937 ) ) ;
#32130=ORIENTED_EDGE ( 'NONE', *, *, #4353, .F. ) ;
#32131=ORIENTED_EDGE ( 'NONE', *, *, #87210, .T. ) ;
#32132=EDGE_CURVE ( 'NONE', #105289, #38108, #2859, .T. ) ;
#32133=DIRECTION ( 'NONE',  ( -0.000000000000000000, 1.000000000000000000, -0.000000000000000000 ) ) ;
#32134=DIRECTION ( 'NONE',  ( 0.000000000000000000, 0.000000000000000000, 1.000000000000000000 ) ) ;
#32135=CIRCLE ( 'NONE', #28191, 0.06509327318403745899 ) ;
#32137=DIRECTION ( 'NONE',  ( -0.000000000000000000, 1.000000000000000000, -0.000000000000000000 ) ) ;
#32138=CARTESIAN_POINT ( 'NONE',  ( -9.800000000000004263, 12.50000000000000000, 3.983716857408420076 ) ) ;
#32139=CONICAL_SURFACE ( 'NONE', #48856, 0.09999999999999982514, 0.003490658503988666988 ) ;
#32140=CARTESIAN_POINT ( 'NONE',  ( 9.599999999999914380, 2.500000000000000000, -4.330127018922201643 ) ) ;
#32141=AXIS2_PLACEMENT_3D ( 'NONE', #53630, #20946, #11763 ) ;
#32142=VECTOR ( 'NONE', #48848, 1000.000000000000000 ) ;
#32143=CARTESIAN_POINT ( 'NONE',  ( -5.400000000000020783, 2.500000000000000000, 5.022947341949748790 ) ) ;
#32144=VERTEX_POINT ( 'NONE', #34274 ) ;
#32145=CIRCLE ( 'NONE', #105280, 0.09999999999999982514 ) ;
#32146=AXIS2_PLACEMENT_3D ( 'NONE', #85314, #63754, #53928 ) ;
#32147=ORIENTED_EDGE ( 'NONE', *, *, #54304, .F. ) ;
#32148=ORIENTED_EDGE ( 'NONE', *, *, #11583, .F. ) ;
#32149=ORIENTED_EDGE ( 'NONE', *, *, #110141, .T. ) ;
#32150=ORIENTED_EDGE ( 'NONE', *, *, #103710, .F. ) ;
#32151=DIRECTION ( 'NONE',  ( -0.000000000000000000, 1.000000000000000000, -0.000000000000000000 ) ) ;
#32152=DIRECTION ( 'NONE',  ( -0.000000000000000000, 1.000000000000000000, -0.000000000000000000 ) ) ;
#32153=DIRECTION ( 'NONE',  ( 0.000000000000000000, 0.000000000000000000, -1.000000000000000000 ) ) ;
#32154=CARTESIAN_POINT ( 'NONE',  ( -8.350000000000013856, 2.500000000000000000, -2.165063509461101710 ) ) ;
#32155=LINE ( 'NONE', #49862, #40965 ) ;
#32156=ORIENTED_EDGE ( 'NONE', *, *, #86084, .F. ) ;
#32157=FACE_OUTER_BOUND ( 'NONE', #109105, .T. ) ;
#32158=LINE ( 'NONE', #123715, #26456 ) ;
#32159=CIRCLE ( 'NONE', #117897, 0.09999999999999982514 ) ;
#32160=AXIS2_PLACEMENT_3D ( 'NONE', #45112, #15622, #53635 ) ;
#32161=DIRECTION ( 'NONE',  ( 0.000000000000000000, 0.000000000000000000, -1.000000000000000000 ) ) ;
#32162=DIRECTION ( 'NONE',  ( 0.000000000000000000, -0.000000000000000000, 1.000000000000000000 ) ) ;
#32163=DIRECTION ( 'NONE',  ( -0.000000000000000000, -1.000000000000000000, -0.000000000000000000 ) ) ;
#32164=VERTEX_POINT ( 'NONE', #52597 ) ;
#32165=CIRCLE ( 'NONE', #90627, 0.06509327318403745899 ) ;
#32166=VECTOR ( 'NONE', #47593, 1000.000000000000000 ) ;
#32167=AXIS2_PLACEMENT_3D ( 'NONE', #3867, #14317, #94181 ) ;
#32168=ORIENTED_EDGE ( 'NONE', *, *, #174, .F. ) ;
#32169=AXIS2_PLACEMENT_3D ( 'NONE', #67147, #59323, #18724 ) ;
#32170=VERTEX_POINT ( 'NONE', #111523 ) ;
#32171=AXIS2_PLACEMENT_3D ( 'NONE', #83953, #23769, #124546 ) ;
#32172=EDGE_CURVE ( 'NONE', #1525, #41325, #29642, .T. ) ;
#32173=CARTESIAN_POINT ( 'NONE',  ( 11.64999999999990798, 12.50000000000000000, -1.472243186433550122 ) ) ;
#32174=EDGE_CURVE ( 'NONE', #81531, #26010, #4564, .T. ) ;
#32175=EDGE_CURVE ( 'NONE', #91490, #80874, #38058, .T. ) ;
#32176=EDGE_LOOP ( 'NONE', ( #120091, #8624, #11970, #103363 ) ) ;
#32177=DIRECTION ( 'NONE',  ( -0.000000000000000000, -1.000000000000000000, -0.000000000000000000 ) ) ;
#32178=CARTESIAN_POINT ( 'NONE',  ( 8.299999999999922551, 2.500000000000000000, 4.430127018922196847 ) ) ;
#32179=CONICAL_SURFACE ( 'NONE', #78229, 0.09999999999999982514, 0.003490658503988666988 ) ;
#32180=AXIS2_PLACEMENT_3D ( 'NONE', #77433, #95148, #65010 ) ;
#32181=EDGE_CURVE ( 'NONE', #91773, #119162, #112175, .T. ) ;
#32182=VECTOR ( 'NONE', #5222, 1000.000000000000000 ) ;
#32183=ORIENTED_EDGE ( 'NONE', *, *, #66666, .F. ) ;
#32184=CARTESIAN_POINT ( 'NONE',  ( 11.69999999999990514, 12.50000000000000000, -2.276824562219559311E-15 ) ) ;
#32187=LINE ( 'NONE', #10567, #99873 ) ;
#32188=ADVANCED_FACE ( 'NONE', ( #44072 ), #127933, .T. ) ;
#32189=EDGE_CURVE ( 'NONE', #23353, #75521, #8787, .T. ) ;
#32190=CARTESIAN_POINT ( 'NONE',  ( 10.39999999999991154, 12.50000000000000000, -5.022947341949754119 ) ) ;
#32191=ORIENTED_EDGE ( 'NONE', *, *, #125670, .T. ) ;
#32192=ORIENTED_EDGE ( 'NONE', *, *, #59750, .T. ) ;
#32193=CARTESIAN_POINT ( 'NONE',  ( -7.700000000000016165, 2.500000000000000000, -4.083716857408426826 ) ) ;
#32194=CARTESIAN_POINT ( 'NONE',  ( -8.750000000000007105, 2.500000000000000000, 7.288010851410849256 ) ) ;
#32195=EDGE_CURVE ( 'NONE', #93758, #100479, #98674, .T. ) ;
#32196=CARTESIAN_POINT ( 'NONE',  ( -8.100000000000013856, 2.500000000000000000, -4.676537180435977881 ) ) ;
#32197=AXIS2_PLACEMENT_3D ( 'NONE', #34121, #83220, #24291 ) ;
#32198=CARTESIAN_POINT ( 'NONE',  ( 4.549999999999937650, 12.50000000000000000, 2.165063509461097713 ) ) ;
#32199=VERTEX_POINT ( 'NONE', #83980 ) ;
#32200=ORIENTED_EDGE ( 'NONE', *, *, #23724, .T. ) ;
#32201=DIRECTION ( 'NONE',  ( 0.000000000000000000, -0.9999939076577903929, 0.003490651415223739937 ) ) ;
#32202=DIRECTION ( 'NONE',  ( 0.000000000000000000, 1.000000000000000000, 0.000000000000000000 ) ) ;
#32203=CARTESIAN_POINT ( 'NONE',  ( 6.249999999999932498, 12.50000000000000000, 5.867463478539781896 ) ) ;
#32204=DIRECTION ( 'NONE',  ( -0.000000000000000000, -1.000000000000000000, -0.000000000000000000 ) ) ;
#32205=ORIENTED_EDGE ( 'NONE', *, *, #102164, .F. ) ;
#32206=CIRCLE ( 'NONE', #117941, 0.06509327318403745899 ) ;
#32207=AXIS2_PLACEMENT_3D ( 'NONE', #64850, #45878, #87067 ) ;
#32208=CARTESIAN_POINT ( 'NONE',  ( 5.449999999999936229, 2.500000000000000000, 6.495190528383297135 ) ) ;
#32209=DIRECTION ( 'NONE',  ( 0.000000000000000000, 0.000000000000000000, -1.000000000000000000 ) ) ;
#32210=ORIENTED_EDGE ( 'NONE', *, *, #116704, .F. ) ;
#32211=CARTESIAN_POINT ( 'NONE',  ( -15.59999999999998010, 12.50000000000000000, 0.3464101615137759604 ) ) ;
#32213=ORIENTED_EDGE ( 'NONE', *, *, #112319, .F. ) ;
#32214=FACE_OUTER_BOUND ( 'NONE', #69596, .T. ) ;
#32215=AXIS2_PLACEMENT_3D ( 'NONE', #61882, #12110, #1641 ) ;
#32216=AXIS2_PLACEMENT_3D ( 'NONE', #63873, #102507, #55342 ) ;
#32217=ORIENTED_EDGE ( 'NONE', *, *, #28255, .F. ) ;
#32218=CARTESIAN_POINT ( 'NONE',  ( -10.40000000000000213, 2.500000000000000000, -5.022947341949749678 ) ) ;
#32219=PLANE ( 'NONE',  #64720 ) ;
#32220=EDGE_LOOP ( 'NONE', ( #25564, #60565 ) ) ;
#32221=EDGE_LOOP ( 'NONE', ( #78653, #27595 ) ) ;
#32222=CARTESIAN_POINT ( 'NONE',  ( -1.450000000000035927, 2.500000000000000000, -1.818653347947326138 ) ) ;
#32223=PLANE ( 'NONE',  #14220 ) ;
#32224=DIRECTION ( 'NONE',  ( -0.000000000000000000, -1.000000000000000000, -0.000000000000000000 ) ) ;
#32226=EDGE_CURVE ( 'NONE', #17587, #59274, #36003, .T. ) ;
#32227=CIRCLE ( 'NONE', #88642, 0.06509327318403745899 ) ;
#32228=CARTESIAN_POINT ( 'NONE',  ( -1.050000000000037792, 2.500000000000000000, 1.718653347947321386 ) ) ;
#32229=AXIS2_PLACEMENT_3D ( 'NONE', #103378, #33368, #3247 ) ;
#32230=CIRCLE ( 'NONE', #120044, 0.06509327318403745899 ) ;
#32231=DIRECTION ( 'NONE',  ( 0.000000000000000000, 0.000000000000000000, 1.000000000000000000 ) ) ;
#32232=LINE ( 'NONE', #1448, #40524 ) ;
#32233=DIRECTION ( 'NONE',  ( -4.274815082592931898E-19, -0.9999939076577903929, -0.003490651415223739937 ) ) ;
#32234=VECTOR ( 'NONE', #66335, 1000.000000000000000 ) ;
#32235=DIRECTION ( 'NONE',  ( 0.000000000000000000, 0.000000000000000000, 1.000000000000000000 ) ) ;
#32236=CIRCLE ( 'NONE', #99123, 0.06509327318403745899 ) ;
#32237=VERTEX_POINT ( 'NONE', #33615 ) ;
#32238=EDGE_LOOP ( 'NONE', ( #57949, #107064, #25887, #35666 ) ) ;
#32239=CARTESIAN_POINT ( 'NONE',  ( 11.24999999999990763, 2.500000000000000000, 1.372243186433545370 ) ) ;
#32240=ORIENTED_EDGE ( 'NONE', *, *, #61840, .T. ) ;
#32241=CARTESIAN_POINT ( 'NONE',  ( 0.4499999999999569344, 2.500000000000000000, 2.065063509461097624 ) ) ;
#32242=DIRECTION ( 'NONE',  ( -4.274815082592931898E-19, -0.9999939076577903929, -0.003490651415223739937 ) ) ;
#32243=CARTESIAN_POINT ( 'NONE',  ( 6.649999999999928413, 2.500000000000000000, 2.857883832488649301 ) ) ;
#32244=ORIENTED_EDGE ( 'NONE', *, *, #100437, .F. ) ;
#32245=ORIENTED_EDGE ( 'NONE', *, *, #23518, .F. ) ;
#32246=FACE_BOUND ( 'NONE', #129202, .T. ) ;
#32247=EDGE_LOOP ( 'NONE', ( #62880, #57489, #112907, #72102 ) ) ;
#32248=DIRECTION ( 'NONE',  ( 0.000000000000000000, 1.000000000000000000, 0.000000000000000000 ) ) ;
#32249=CARTESIAN_POINT ( 'NONE',  ( 2.099999999999948574, 2.500000000000000000, 3.537306695894645081 ) ) ;
#32250=DIRECTION ( 'NONE',  ( -0.000000000000000000, 1.000000000000000000, -0.000000000000000000 ) ) ;
#32251=DIRECTION ( 'NONE',  ( 0.000000000000000000, 1.000000000000000000, 0.000000000000000000 ) ) ;
#32253=DIRECTION ( 'NONE',  ( 0.000000000000000000, 0.000000000000000000, 1.000000000000000000 ) ) ;
#32254=CIRCLE ( 'NONE', #69883, 0.1000000000000002554 ) ;
#32255=DIRECTION ( 'NONE',  ( -0.000000000000000000, -1.000000000000000000, -0.000000000000000000 ) ) ;
#32256=LINE ( 'NONE', #72170, #58930 ) ;
#32257=CIRCLE ( 'NONE', #42726, 0.1000000000000000472 ) ;
#32258=CIRCLE ( 'NONE', #124269, 0.1000000000000002554 ) ;
#32259=DIRECTION ( 'NONE',  ( 0.000000000000000000, 1.000000000000000000, 0.000000000000000000 ) ) ;
#32260=DIRECTION ( 'NONE',  ( -0.000000000000000000, 1.000000000000000000, -0.000000000000000000 ) ) ;
#32261=PLANE ( 'NONE',  #66035 ) ;
#32263=ORIENTED_EDGE ( 'NONE', *, *, #111349, .F. ) ;
#32264=EDGE_LOOP ( 'NONE', ( #12272, #81124 ) ) ;
#32265=EDGE_LOOP ( 'NONE', ( #56531, #121630 ) ) ;
#32266=CONICAL_SURFACE ( 'NONE', #90732, 0.1000000000000002554, 0.003490658503988666988 ) ;
#32267=CARTESIAN_POINT ( 'NONE',  ( 12.09999999999990195, 2.500000000000000000, -2.276824562219559311E-15 ) ) ;
#32268=ORIENTED_EDGE ( 'NONE', *, *, #111642, .F. ) ;
#32269=DIRECTION ( 'NONE',  ( 0.000000000000000000, 0.000000000000000000, 1.000000000000000000 ) ) ;
#32270=DIRECTION ( 'NONE',  ( -0.000000000000000000, -1.000000000000000000, -0.000000000000000000 ) ) ;
#32271=EDGE_LOOP ( 'NONE', ( #41046, #17696, #88270, #18279 ) ) ;
#32272=ORIENTED_EDGE ( 'NONE', *, *, #44533, .F. ) ;
#32273=ORIENTED_EDGE ( 'NONE', *, *, #81346, .F. ) ;
#32274=DIRECTION ( 'NONE',  ( 0.000000000000000000, 0.000000000000000000, 1.000000000000000000 ) ) ;
#32275=CIRCLE ( 'NONE', #105407, 0.06509327318403745899 ) ;
#32276=AXIS2_PLACEMENT_3D ( 'NONE', #100306, #10600, #50538 ) ;
#32277=ADVANCED_FACE ( 'NONE', ( #123913 ), #96513, .T. ) ;
#32278=CARTESIAN_POINT ( 'NONE',  ( -0.4000000000000396572, 2.500000000000000000, 4.330127018922196314 ) ) ;
#32279=SHAPE_REPRESENTATION_RELATIONSHIP ( 'NONE' , 'NONE' ,  #1094, #119481 ) ;
#32280=DIRECTION ( 'NONE',  ( 0.000000000000000000, 0.000000000000000000, 1.000000000000000000 ) ) ;
#32281=DIRECTION ( 'NONE',  ( 0.000000000000000000, -0.9999939076577903929, 0.003490651415223739937 ) ) ;
#32282=FACE_OUTER_BOUND ( 'NONE', #54050, .T. ) ;
#32283=AXIS2_PLACEMENT_3D ( 'NONE', #114379, #3160, #42443 ) ;
#32284=DIRECTION ( 'NONE',  ( 0.000000000000000000, 0.000000000000000000, 1.000000000000000000 ) ) ;
#32285=EDGE_CURVE ( 'NONE', #37178, #88690, #21317, .T. ) ;
#32286=ORIENTED_EDGE ( 'NONE', *, *, #14435, .F. ) ;
#32287=EDGE_CURVE ( 'NONE', #30841, #74045, #64353, .T. ) ;
#32288=CARTESIAN_POINT ( 'NONE',  ( 3.149999999999946176, 2.500000000000000000, -2.511473670974877948 ) ) ;
#32289=VERTEX_POINT ( 'NONE', #91888 ) ;
#32290=VERTEX_POINT ( 'NONE', #12024 ) ;
#32291=ORIENTED_EDGE ( 'NONE', *, *, #84446, .F. ) ;
#32292=EDGE_CURVE ( 'NONE', #32739, #17445, #94468, .T. ) ;
#32293=FACE_OUTER_BOUND ( 'NONE', #20036, .T. ) ;
#32294=ADVANCED_FACE ( 'NONE', ( #72261 ), #117431, .T. ) ;
#32295=EDGE_CURVE ( 'NONE', #6764, #88013, #102360, .T. ) ;
#32296=VERTEX_POINT ( 'NONE', #112821 ) ;
#32297=EDGE_LOOP ( 'NONE', ( #93048, #125556, #106215, #85508 ) ) ;
#32298=ADVANCED_FACE ( 'NONE', ( #102984 ), #46354, .T. ) ;
#32299=ADVANCED_FACE ( 'NONE', ( #43450 ), #106984, .T. ) ;
#32300=ORIENTED_EDGE ( 'NONE', *, *, #2219, .F. ) ;
#32301=VECTOR ( 'NONE', #89019, 1000.000000000000000 ) ;
#32302=DIRECTION ( 'NONE',  ( 0.000000000000000000, 1.000000000000000000, 0.000000000000000000 ) ) ;
#32303=DIRECTION ( 'NONE',  ( 0.000000000000000000, 0.000000000000000000, 1.000000000000000000 ) ) ;
#32304=CARTESIAN_POINT ( 'NONE',  ( 14.14999999999989377, 2.500000000000000000, -2.757883832488654097 ) ) ;
#32305=LINE ( 'NONE', #82680, #8673 ) ;
#32306=CARTESIAN_POINT ( 'NONE',  ( -4.600000000000024514, 2.500000000000000000, 3.637306695894644726 ) ) ;
#32307=CARTESIAN_POINT ( 'NONE',  ( 12.69999999999990159, 2.500000000000000000, -3.983716857408426293 ) ) ;
#32308=EDGE_CURVE ( 'NONE', #55936, #38064, #125863, .T. ) ;
#32309=DIRECTION ( 'NONE',  ( 0.000000000000000000, 0.000000000000000000, 1.000000000000000000 ) ) ;
#32310=CIRCLE ( 'NONE', #57318, 0.06509327318403741736 ) ;
#32311=AXIS2_PLACEMENT_3D ( 'NONE', #30761, #70660, #62789 ) ;
#32312=ORIENTED_EDGE ( 'NONE', *, *, #89307, .F. ) ;
#32313=CARTESIAN_POINT ( 'NONE',  ( -1.850000000000033396, 2.500000000000000000, -6.741600689897077281 ) ) ;
#32314=VERTEX_POINT ( 'NONE', #6060 ) ;
#32315=CARTESIAN_POINT ( 'NONE',  ( 3.099999999999945022, 2.500000000000000000, -4.676537180435978769 ) ) ;
#32316=ORIENTED_EDGE ( 'NONE', *, *, #69202, .T. ) ;
#32317=DIRECTION ( 'NONE',  ( 0.000000000000000000, 0.000000000000000000, 1.000000000000000000 ) ) ;
#32318=VERTEX_POINT ( 'NONE', #86564 ) ;
#32319=DIRECTION ( 'NONE',  ( 0.000000000000000000, 0.000000000000000000, 1.000000000000000000 ) ) ;
#32320=CIRCLE ( 'NONE', #11358, 0.1000000000000002554 ) ;
#32321=CARTESIAN_POINT ( 'NONE',  ( 4.999999999999969802, 2.500000000000000000, 4.430127018922196847 ) ) ;
#32322=ORIENTED_EDGE ( 'NONE', *, *, #129062, .F. ) ;
#32323=VERTEX_POINT ( 'NONE', #46654 ) ;
#32324=CARTESIAN_POINT ( 'NONE',  ( 2.699999999999946443, 12.50000000000000000, -3.983716857408426293 ) ) ;
#32325=LINE ( 'NONE', #62416, #95403 ) ;
#32326=CARTESIAN_POINT ( 'NONE',  ( 15.39999999999989200, 12.50000000000000000, 0.6277270498435120194 ) ) ;
#32327=LINE ( 'NONE', #42796, #40941 ) ;
#32328=FACE_OUTER_BOUND ( 'NONE', #101610, .T. ) ;
#32329=ORIENTED_EDGE ( 'NONE', *, *, #5841, .T. ) ;
#32330=CIRCLE ( 'NONE', #40644, 0.09999999999999982514 ) ;
#32331=CIRCLE ( 'NONE', #84524, 0.09999999999999999167 ) ;
#32332=DIRECTION ( 'NONE',  ( 0.000000000000000000, 0.000000000000000000, -1.000000000000000000 ) ) ;
#32333=CIRCLE ( 'NONE', #99213, 0.09999999999999999167 ) ;
#32334=EDGE_CURVE ( 'NONE', #47052, #17385, #111191, .T. ) ;
#32335=EDGE_CURVE ( 'NONE', #128936, #740, #56804, .T. ) ;
#32336=VERTEX_POINT ( 'NONE', #57768 ) ;
#32337=AXIS2_PLACEMENT_3D ( 'NONE', #72292, #72922, #70343 ) ;
#32338=DIRECTION ( 'NONE',  ( 0.000000000000000000, 1.000000000000000000, 0.000000000000000000 ) ) ;
#32339=CARTESIAN_POINT ( 'NONE',  ( 9.599999999999917932, 12.50000000000000000, -0.6928203230275541413 ) ) ;
#32340=ADVANCED_FACE ( 'NONE', ( #66916 ), #36200, .T. ) ;
#32342=CARTESIAN_POINT ( 'NONE',  ( 9.599999999999914380, 2.500000000000000000, -3.637306695894650055 ) ) ;
#32343=DIRECTION ( 'NONE',  ( -0.000000000000000000, 1.000000000000000000, -0.000000000000000000 ) ) ;
#32344=EDGE_CURVE ( 'NONE', #4941, #121191, #73539, .T. ) ;
#32345=CARTESIAN_POINT ( 'NONE',  ( -8.100000000000013856, 2.500000000000000000, -4.676537180435977881 ) ) ;
#32346=DIRECTION ( 'NONE',  ( 0.000000000000000000, 1.000000000000000000, 0.000000000000000000 ) ) ;
#32347=ORIENTED_EDGE ( 'NONE', *, *, #124515, .F. ) ;
#32348=EDGE_CURVE ( 'NONE', #19669, #87504, #54760, .T. ) ;
#32349=EDGE_CURVE ( 'NONE', #91045, #32427, #123705, .T. ) ;
#32350=DIRECTION ( 'NONE',  ( 0.000000000000000000, 1.000000000000000000, 0.000000000000000000 ) ) ;
#32351=EDGE_CURVE ( 'NONE', #98420, #48878, #10834, .T. ) ;
#32352=DIRECTION ( 'NONE',  ( 0.000000000000000000, 0.000000000000000000, 1.000000000000000000 ) ) ;
#32353=DIRECTION ( 'NONE',  ( 0.000000000000000000, -0.9999939076577903929, 0.003490651415223739937 ) ) ;
#32354=CIRCLE ( 'NONE', #69981, 0.1000000000000002554 ) ;
#32355=ORIENTED_EDGE ( 'NONE', *, *, #45302, .T. ) ;
#32356=CIRCLE ( 'NONE', #40753, 0.1000000000000002554 ) ;
#32357=AXIS2_PLACEMENT_3D ( 'NONE', #86802, #118841, #117522 ) ;
#32358=ORIENTED_EDGE ( 'NONE', *, *, #64205, .F. ) ;
#32359=EDGE_CURVE ( 'NONE', #70177, #12234, #90259, .T. ) ;
#32360=CARTESIAN_POINT ( 'NONE',  ( -9.350000000000006750, 12.50000000000000000, 2.511473670974873507 ) ) ;
#32361=AXIS2_PLACEMENT_3D ( 'NONE', #31318, #98097, #8419 ) ;
#32362=VECTOR ( 'NONE', #108691, 1000.000000000000000 ) ;
#32363=EDGE_LOOP ( 'NONE', ( #28364, #26872 ) ) ;
#32364=AXIS2_PLACEMENT_3D ( 'NONE', #72368, #83479, #52079 ) ;
#32365=ORIENTED_EDGE ( 'NONE', *, *, #19158, .F. ) ;
#32366=FACE_OUTER_BOUND ( 'NONE', #110659, .T. ) ;
#32367=CIRCLE ( 'NONE', #72349, 0.1000000000000000472 ) ;
#32368=ORIENTED_EDGE ( 'NONE', *, *, #73503, .F. ) ;
#32369=CARTESIAN_POINT ( 'NONE',  ( 16.79927703353608592, -2.472530191752320139, -3.248144252806293597 ) ) ;
#32370=FACE_OUTER_BOUND ( 'NONE', #85186, .T. ) ;
#32371=CARTESIAN_POINT ( 'NONE',  ( 8.349999999999923261, 2.500000000000000000, -7.188010851410854052 ) ) ;
#32372=VERTEX_POINT ( 'NONE', #66288 ) ;
#32373=CONICAL_SURFACE ( 'NONE', #105506, 0.09999999999999982514, 0.003490658503988666988 ) ;
#32374=CONICAL_SURFACE ( 'NONE', #26088, 0.1000000000000000472, 0.003490658503988666988 ) ;
#32375=CARTESIAN_POINT ( 'NONE',  ( 5.649999999999934630, 2.500000000000000000, -1.818653347947325916 ) ) ;
#32376=DIRECTION ( 'NONE',  ( 0.000000000000000000, 0.000000000000000000, 1.000000000000000000 ) ) ;
#32377=AXIS2_PLACEMENT_3D ( 'NONE', #18762, #91373, #50814 ) ;
#32378=EDGE_CURVE ( 'NONE', #93110, #9428, #27567, .T. ) ;
#32379=EDGE_LOOP ( 'NONE', ( #12427, #49517 ) ) ;
#32380=VERTEX_POINT ( 'NONE', #34921 ) ;
#32381=ORIENTED_EDGE ( 'NONE', *, *, #74680, .F. ) ;
#32382=DIRECTION ( 'NONE',  ( 0.000000000000000000, 1.000000000000000000, 0.000000000000000000 ) ) ;
#32383=DIRECTION ( 'NONE',  ( -0.000000000000000000, 1.000000000000000000, -0.000000000000000000 ) ) ;
#32384=CARTESIAN_POINT ( 'NONE',  ( -4.150000000000027889, 2.500000000000000000, -7.188010851410854052 ) ) ;
#32385=FACE_BOUND ( 'NONE', #94494, .T. ) ;
#32386=ORIENTED_EDGE ( 'NONE', *, *, #83379, .F. ) ;
#32387=DIRECTION ( 'NONE',  ( -4.274815082592931898E-19, -0.9999939076577903929, -0.003490651415223739937 ) ) ;
#32388=DIRECTION ( 'NONE',  ( 0.000000000000000000, 1.000000000000000000, 0.000000000000000000 ) ) ;
#32389=AXIS2_PLACEMENT_3D ( 'NONE', #1050, #41009, #109726 ) ;
#32390=ORIENTED_EDGE ( 'NONE', *, *, #57138, .T. ) ;
#32391=DIRECTION ( 'NONE',  ( 0.000000000000000000, 1.000000000000000000, 0.000000000000000000 ) ) ;
#32392=DIRECTION ( 'NONE',  ( -0.000000000000000000, -1.000000000000000000, -0.000000000000000000 ) ) ;
#32393=ADVANCED_FACE ( 'NONE', ( #105574 ), #44303, .T. ) ;
#32394=DIRECTION ( 'NONE',  ( -4.274815082592931898E-19, -0.9999939076577903929, -0.003490651415223739937 ) ) ;
#32395=DIRECTION ( 'NONE',  ( -0.000000000000000000, 1.000000000000000000, -0.000000000000000000 ) ) ;
#32396=DIRECTION ( 'NONE',  ( -4.274815082592931898E-19, -0.9999939076577903929, -0.003490651415223739937 ) ) ;
#32397=CARTESIAN_POINT ( 'NONE',  ( -6.850000000000017408, 12.50000000000000000, -6.776507416713039689 ) ) ;
#32398=CARTESIAN_POINT ( 'NONE',  ( -4.400000000000028777, 12.50000000000000000, -4.676537180435978769 ) ) ;
#32399=CIRCLE ( 'NONE', #49109, 0.09999999999999982514 ) ;
#32400=ORIENTED_EDGE ( 'NONE', *, *, #125202, .F. ) ;
#32401=VERTEX_POINT ( 'NONE', #8002 ) ;
#32402=ORIENTED_EDGE ( 'NONE', *, *, #26123, .F. ) ;
#32403=VERTEX_POINT ( 'NONE', #17146 ) ;
#32404=FACE_OUTER_BOUND ( 'NONE', #10196, .T. ) ;
#32405=CARTESIAN_POINT ( 'NONE',  ( -1.250000000000036193, 2.500000000000000000, 5.702370205355745014 ) ) ;
#32406=LINE ( 'NONE', #43498, #105374 ) ;
#32407=ORIENTED_EDGE ( 'NONE', *, *, #6989, .T. ) ;
#32408=ADVANCED_FACE ( 'NONE', ( #64982 ), #81953, .T. ) ;
#32409=FACE_BOUND ( 'NONE', #46725, .T. ) ;
#32410=CARTESIAN_POINT ( 'NONE',  ( 1.249999999999954259, 2.500000000000000000, -7.088010851410853519 ) ) ;
#32411=CARTESIAN_POINT ( 'NONE',  ( -15.39999999999997904, 2.500000000000000000, -0.1000000000000000056 ) ) ;
#32412=CIRCLE ( 'NONE', #101343, 0.06509327318403745899 ) ;
#32413=CARTESIAN_POINT ( 'NONE',  ( -11.25000000000000178, 2.500000000000000000, -1.472243186433546125 ) ) ;
#32414=CARTESIAN_POINT ( 'NONE',  ( -13.34999999999999076, 2.500000000000000000, -2.757883832488651876 ) ) ;
#32415=AXIS2_PLACEMENT_3D ( 'NONE', #92921, #43179, #83097 ) ;
#32416=CARTESIAN_POINT ( 'NONE',  ( -4.400000000000025224, 2.500000000000000000, -0.4464101615137783252 ) ) ;
#32417=LINE ( 'NONE', #23196, #28727 ) ;
#32418=LINE ( 'NONE', #91301, #100091 ) ;
#32419=FACE_OUTER_BOUND ( 'NONE', #117099, .T. ) ;
#32420=CARTESIAN_POINT ( 'NONE',  ( 1.699999999999951994, 2.500000000000000000, -0.1000000000000022815 ) ) ;
#32421=VERTEX_POINT ( 'NONE', #95753 ) ;
#32422=AXIS2_PLACEMENT_3D ( 'NONE', #77892, #98184, #8501 ) ;
#32423=ORIENTED_EDGE ( 'NONE', *, *, #4401, .T. ) ;
#32425=AXIS2_PLACEMENT_3D ( 'NONE', #70372, #110296, #118826 ) ;
#32426=ORIENTED_EDGE ( 'NONE', *, *, #47669, .T. ) ;
#32427=VERTEX_POINT ( 'NONE', #97040 ) ;
#32428=ORIENTED_EDGE ( 'NONE', *, *, #98186, .F. ) ;
#32429=DIRECTION ( 'NONE',  ( 0.000000000000000000, 0.000000000000000000, 1.000000000000000000 ) ) ;
#32430=EDGE_LOOP ( 'NONE', ( #8798, #18461, #71265, #45800 ) ) ;
#32431=ORIENTED_EDGE ( 'NONE', *, *, #81915, .F. ) ;
#32432=CIRCLE ( 'NONE', #128575, 0.09999999999999999167 ) ;
#32433=EDGE_CURVE ( 'NONE', #15887, #76186, #15229, .T. ) ;
#32434=CARTESIAN_POINT ( 'NONE',  ( -3.350000000000029399, 12.50000000000000000, 6.430097255199259010 ) ) ;
#32435=CARTESIAN_POINT ( 'NONE',  ( 15.50668943717099602, -1.500000000000000222, 6.997696160023530787 ) ) ;
#32436=CARTESIAN_POINT ( 'NONE',  ( -10.45000000000000107, 2.500000000000000000, 2.165063509461097713 ) ) ;
#32437=CARTESIAN_POINT ( 'NONE',  ( 7.699999999999923794, 2.500000000000000000, -0.4464101615137783252 ) ) ;
#32438=ORIENTED_EDGE ( 'NONE', *, *, #104165, .T. ) ;
#32439=CARTESIAN_POINT ( 'NONE',  ( -3.749999999999991118, 2.500000000000000000, 2.165063509461097713 ) ) ;
#32440=ORIENTED_EDGE ( 'NONE', *, *, #128230, .F. ) ;
#32441=AXIS2_PLACEMENT_3D ( 'NONE', #115826, #56260, #7147 ) ;
#32442=ORIENTED_EDGE ( 'NONE', *, *, #74417, .F. ) ;
#32443=FACE_OUTER_BOUND ( 'NONE', #34162, .T. ) ;
#32444=CIRCLE ( 'NONE', #78498, 0.09999999999999982514 ) ;
#32445=EDGE_CURVE ( 'NONE', #30581, #80023, #75688, .T. ) ;
#32446=DIRECTION ( 'NONE',  ( 0.000000000000000000, 0.000000000000000000, 1.000000000000000000 ) ) ;
#32447=EDGE_CURVE ( 'NONE', #80892, #110135, #92421, .T. ) ;
#32448=EDGE_CURVE ( 'NONE', #45085, #58857, #35555, .T. ) ;
#32449=ADVANCED_FACE ( 'NONE', ( #25714 ), #62770, .T. ) ;
#32450=ORIENTED_EDGE ( 'NONE', *, *, #98439, .F. ) ;
#32451=ORIENTED_EDGE ( 'NONE', *, *, #29259, .F. ) ;
#32452=DIRECTION ( 'NONE',  ( 0.000000000000000000, 0.000000000000000000, 1.000000000000000000 ) ) ;
#32453=AXIS2_PLACEMENT_3D ( 'NONE', #15507, #25998, #65902 ) ;
#32454=CONICAL_SURFACE ( 'NONE', #74188, 0.09999999999999982514, 0.003490658503988666988 ) ;
#32455=AXIS2_PLACEMENT_3D ( 'NONE', #30364, #70275, #63025 ) ;
#32456=PLANE ( 'NONE',  #114312 ) ;
#32457=DIRECTION ( 'NONE',  ( -4.274815082592931898E-19, -0.9999939076577903929, -0.003490651415223739937 ) ) ;
#32458=DIRECTION ( 'NONE',  ( 0.000000000000000000, -0.000000000000000000, 1.000000000000000000 ) ) ;
#32459=CARTESIAN_POINT ( 'NONE',  ( -2.050000000000032685, 12.50000000000000000, -6.495190528383302464 ) ) ;
#32460=EDGE_CURVE ( 'NONE', #82094, #120092, #43990, .T. ) ;
#32461=VERTEX_POINT ( 'NONE', #41841 ) ;
#32462=DIRECTION ( 'NONE',  ( -0.000000000000000000, 1.000000000000000000, -0.000000000000000000 ) ) ;
#32463=ADVANCED_FACE ( 'NONE', ( #70634 ), #77422, .T. ) ;
#32464=CIRCLE ( 'NONE', #28322, 0.06509327318403745899 ) ;
#32465=VECTOR ( 'NONE', #96436, 1000.000000000000000 ) ;
#32467=ORIENTED_EDGE ( 'NONE', *, *, #107874, .T. ) ;
#32468=LINE ( 'NONE', #34388, #81705 ) ;
#32469=CARTESIAN_POINT ( 'NONE',  ( 7.099999999999927702, 12.50000000000000000, 4.957854068765711553 ) ) ;
#32470=CARTESIAN_POINT ( 'NONE',  ( -9.150000000000009237, 12.50000000000000000, -7.188010851410848723 ) ) ;
#32471=CIRCLE ( 'NONE', #40871, 0.06509327318403745899 ) ;
#32472=DIRECTION ( 'NONE',  ( 0.000000000000000000, 0.000000000000000000, 1.000000000000000000 ) ) ;
#32474=ORIENTED_EDGE ( 'NONE', *, *, #105422, .F. ) ;
#32475=CARTESIAN_POINT ( 'NONE',  ( 10.59999999999990905, 2.500000000000000000, 3.983716857408420076 ) ) ;
#32476=DIRECTION ( 'NONE',  ( -4.274815082592931898E-19, -0.9999939076577903929, -0.003490651415223739937 ) ) ;
#32477=ORIENTED_EDGE ( 'NONE', *, *, #83562, .F. ) ;
#32479=ORIENTED_EDGE ( 'NONE', *, *, #973, .F. ) ;
#32480=FACE_OUTER_BOUND ( 'NONE', #20954, .T. ) ;
#32481=CARTESIAN_POINT ( 'NONE',  ( -0.2000000000000408673, 2.500000000000000000, -3.983716857408426293 ) ) ;
#32483=AXIS2_PLACEMENT_3D ( 'NONE', #40110, #158, #78761 ) ;
#32484=CARTESIAN_POINT ( 'NONE',  ( -0.4000000000000331624, 2.500000000000000000, -0.7928203230275518987 ) ) ;
#32485=PLANE ( 'NONE',  #31995 ) ;
#32486=CARTESIAN_POINT ( 'NONE',  ( 17.01005371150552037, 1.931450858213933808, -5.528361852685595323 ) ) ;
#32487=CARTESIAN_POINT ( 'NONE',  ( -12.09999999999999432, 12.50000000000000000, 3.702399969078682407 ) ) ;
#32488=CONICAL_SURFACE ( 'NONE', #49208, 0.1000000000000000472, 0.003490658503988666988 ) ;
#32489=CIRCLE ( 'NONE', #51356, 0.06509327318403745899 ) ;
#32490=DIRECTION ( 'NONE',  ( -0.000000000000000000, -1.000000000000000000, -0.000000000000000000 ) ) ;
#32491=ORIENTED_EDGE ( 'NONE', *, *, #34902, .T. ) ;
#32492=CARTESIAN_POINT ( 'NONE',  ( -7.500000000000016875, 12.50000000000000000, -3.637306695894650055 ) ) ;
#32493=DIRECTION ( 'NONE',  ( -0.000000000000000000, -1.000000000000000000, -0.000000000000000000 ) ) ;
#32494=CARTESIAN_POINT ( 'NONE',  ( 11.69999999999990870, 2.500000000000000000, 4.230127018922196669 ) ) ;
#32495=DIRECTION ( 'NONE',  ( 0.000000000000000000, 1.000000000000000000, 0.000000000000000000 ) ) ;
#32496=ORIENTED_EDGE ( 'NONE', *, *, #1401, .F. ) ;
#32497=CARTESIAN_POINT ( 'NONE',  ( -11.64999999999999680, 2.500000000000000000, -2.757883832488650100 ) ) ;
#32498=AXIS2_PLACEMENT_3D ( 'NONE', #41994, #3984, #114581 ) ;
#32499=EDGE_CURVE ( 'NONE', #50102, #11701, #102470, .T. ) ;
#32500=AXIS2_PLACEMENT_3D ( 'NONE', #99360, #77131, #77756 ) ;
#32501=EDGE_CURVE ( 'NONE', #92671, #68126, #70001, .T. ) ;
#32502=CARTESIAN_POINT ( 'NONE',  ( -6.650000000000014566, 2.500000000000000000, 2.165063509461097713 ) ) ;
#32503=FACE_OUTER_BOUND ( 'NONE', #76109, .T. ) ;
#32504=EDGE_LOOP ( 'NONE', ( #78631, #91730, #59060, #68964 ) ) ;
#32505=ORIENTED_EDGE ( 'NONE', *, *, #120188, .F. ) ;
#32506=EDGE_CURVE ( 'NONE', #7114, #104821, #32023, .T. ) ;
#32507=FACE_OUTER_BOUND ( 'NONE', #59547, .T. ) ;
#32509=ORIENTED_EDGE ( 'NONE', *, *, #115026, .T. ) ;
#32510=EDGE_LOOP ( 'NONE', ( #21968, #119216, #24277, #32150 ) ) ;
#32511=DIRECTION ( 'NONE',  ( -0.000000000000000000, -1.000000000000000000, -0.000000000000000000 ) ) ;
#32512=CARTESIAN_POINT ( 'NONE',  ( 19.72570408286475185, 0.6078483229322081405, -4.299616118078707139 ) ) ;
#32514=DIRECTION ( 'NONE',  ( -0.000000000000000000, 1.000000000000000000, -0.000000000000000000 ) ) ;
#32515=VERTEX_POINT ( 'NONE', #22851 ) ;
#32516=CONICAL_SURFACE ( 'NONE', #93146, 0.1000000000000002554, 0.003490658503988666988 ) ;
#32517=PLANE ( 'NONE',  #73391 ) ;
#32518=ORIENTED_EDGE ( 'NONE', *, *, #1132, .F. ) ;
#32519=DIRECTION ( 'NONE',  ( -0.000000000000000000, 1.000000000000000000, -0.000000000000000000 ) ) ;
#32520=DIRECTION ( 'NONE',  ( 0.000000000000000000, 0.000000000000000000, 1.000000000000000000 ) ) ;
#32521=AXIS2_PLACEMENT_3D ( 'NONE', #7783, #77179, #108571 ) ;
#32522=EDGE_LOOP ( 'NONE', ( #95671, #104051, #96966, #88777 ) ) ;
#32523=VECTOR ( 'NONE', #3791, 1000.000000000000000 ) ;
#32524=ORIENTED_EDGE ( 'NONE', *, *, #36285, .F. ) ;
#32525=AXIS2_PLACEMENT_3D ( 'NONE', #36820, #16501, #95087 ) ;
#32526=VERTEX_POINT ( 'NONE', #71942 ) ;
#32527=EDGE_LOOP ( 'NONE', ( #88218, #104356 ) ) ;
#32528=CARTESIAN_POINT ( 'NONE',  ( -0.4500000000000397571, 12.50000000000000000, -2.165063509461101710 ) ) ;
#32529=FACE_OUTER_BOUND ( 'NONE', #78473, .T. ) ;
#32530=CARTESIAN_POINT ( 'NONE',  ( 1.249999999999986899, 12.50000000000000000, 6.495190528383297135 ) ) ;
#32531=FACE_BOUND ( 'NONE', #114633, .T. ) ;
#32532=VERTEX_POINT ( 'NONE', #127783 ) ;
#32534=CARTESIAN_POINT ( 'NONE',  ( 13.94999999999989804, 12.50000000000000000, 1.883746621131358934 ) ) ;
#32535=DIRECTION ( 'NONE',  ( 0.000000000000000000, 0.000000000000000000, 1.000000000000000000 ) ) ;
#32536=AXIS2_PLACEMENT_3D ( 'NONE', #104859, #15182, #55137 ) ;
#32537=VECTOR ( 'NONE', #60473, 1000.000000000000000 ) ;
#32538=ADVANCED_FACE ( 'NONE', ( #62763 ), #12353, .T. ) ;
#32539=CARTESIAN_POINT ( 'NONE',  ( -3.749999999999991562, 12.50000000000000000, 6.430097255199259010 ) ) ;
#32540=CONICAL_SURFACE ( 'NONE', #105681, 0.09999999999999982514, 0.003490658503988666988 ) ;
#32541=DIRECTION ( 'NONE',  ( 0.000000000000000000, 0.000000000000000000, 1.000000000000000000 ) ) ;
#32542=DIRECTION ( 'NONE',  ( -0.000000000000000000, -1.000000000000000000, -0.000000000000000000 ) ) ;
#32543=CONICAL_SURFACE ( 'NONE', #82713, 0.1000000000000002554, 0.003490658503988666988 ) ;
#32544=AXIS2_PLACEMENT_3D ( 'NONE', #10009, #118021, #39498 ) ;
#32545=DIRECTION ( 'NONE',  ( -0.000000000000000000, 1.000000000000000000, -0.000000000000000000 ) ) ;
#32546=CIRCLE ( 'NONE', #20098, 0.06509327318403743123 ) ;
#32547=ORIENTED_EDGE ( 'NONE', *, *, #47179, .F. ) ;
#32548=VERTEX_POINT ( 'NONE', #92200 ) ;
#32549=ORIENTED_EDGE ( 'NONE', *, *, #97306, .F. ) ;
#32550=VERTEX_POINT ( 'NONE', #32678 ) ;
#32551=AXIS2_PLACEMENT_3D ( 'NONE', #71395, #51147, #121792 ) ;
#32552=EDGE_CURVE ( 'NONE', #19348, #84309, #96191, .T. ) ;
#32553=ORIENTED_EDGE ( 'NONE', *, *, #56764, .F. ) ;
#32554=CARTESIAN_POINT ( 'NONE',  ( 7.049999999999928768, 12.50000000000000000, -2.165063509461101710 ) ) ;
#32555=DIRECTION ( 'NONE',  ( 0.000000000000000000, -0.9999939076577903929, 0.003490651415223739937 ) ) ;
#32556=VERTEX_POINT ( 'NONE', #51016 ) ;
#32557=EDGE_CURVE ( 'NONE', #97573, #81547, #31371, .T. ) ;
#32558=FACE_BOUND ( 'NONE', #103368, .T. ) ;
#32559=CARTESIAN_POINT ( 'NONE',  ( -12.29999999999999716, 12.50000000000000000, -3.983716857408423628 ) ) ;
#32560=ORIENTED_EDGE ( 'NONE', *, *, #1089, .F. ) ;
#32561=DIRECTION ( 'NONE',  ( 0.000000000000000000, 1.000000000000000000, 0.000000000000000000 ) ) ;
#32562=ADVANCED_FACE ( 'NONE', ( #41201 ), #110557, .T. ) ;
#32563=DIRECTION ( 'NONE',  ( 0.000000000000000000, -0.000000000000000000, 1.000000000000000000 ) ) ;
#32564=DIRECTION ( 'NONE',  ( -0.000000000000000000, -1.000000000000000000, -0.000000000000000000 ) ) ;
#32565=AXIS2_PLACEMENT_3D ( 'NONE', #107395, #77290, #47848 ) ;
#32566=ORIENTED_EDGE ( 'NONE', *, *, #118111, .F. ) ;
#32567=DIRECTION ( 'NONE',  ( -4.274815082592931898E-19, -0.9999939076577903929, -0.003490651415223739937 ) ) ;
#32568=ORIENTED_EDGE ( 'NONE', *, *, #101453, .T. ) ;
#32569=ORIENTED_EDGE ( 'NONE', *, *, #67280, .T. ) ;
#32570=ORIENTED_EDGE ( 'NONE', *, *, #37525, .F. ) ;
#32571=DIRECTION ( 'NONE',  ( -0.000000000000000000, 1.000000000000000000, -0.000000000000000000 ) ) ;
#32572=CARTESIAN_POINT ( 'NONE',  ( -7.499999999999980460, 12.50000000000000000, -4.330127018922201643 ) ) ;
#32573=CIRCLE ( 'NONE', #111980, 0.06509327318403743123 ) ;
#32574=DIRECTION ( 'NONE',  ( 0.000000000000000000, 1.000000000000000000, 0.000000000000000000 ) ) ;
#32576=DIRECTION ( 'NONE',  ( -4.274815082592931898E-19, -0.9999939076577903929, -0.003490651415223739937 ) ) ;
#32578=VECTOR ( 'NONE', #966, 1000.000000000000000 ) ;
#32579=DIRECTION ( 'NONE',  ( 0.000000000000000000, 0.000000000000000000, 1.000000000000000000 ) ) ;
#32580=CIRCLE ( 'NONE', #28643, 0.1000000000000000472 ) ;
#32581=CARTESIAN_POINT ( 'NONE',  ( 12.89999999999990088, 12.50000000000000000, -4.330127018922201643 ) ) ;
#32582=EDGE_CURVE ( 'NONE', #114322, #10341, #110860, .T. ) ;
#32583=DIRECTION ( 'NONE',  ( -0.000000000000000000, 1.000000000000000000, -0.000000000000000000 ) ) ;
#32584=CARTESIAN_POINT ( 'NONE',  ( -4.150000000000025224, 12.50000000000000000, 6.495190528383297135 ) ) ;
#32585=ORIENTED_EDGE ( 'NONE', *, *, #1089, .T. ) ;
#32586=DIRECTION ( 'NONE',  ( 0.000000000000000000, -0.9999939076577903929, 0.003490651415223739937 ) ) ;
#32587=ORIENTED_EDGE ( 'NONE', *, *, #63171, .F. ) ;
#32588=DIRECTION ( 'NONE',  ( 0.000000000000000000, 1.000000000000000000, 0.000000000000000000 ) ) ;
#32589=CONICAL_SURFACE ( 'NONE', #66006, 0.09999999999999982514, 0.003490658503988666988 ) ;
#32590=EDGE_CURVE ( 'NONE', #22957, #59076, #112933, .T. ) ;
#32591=ORIENTED_EDGE ( 'NONE', *, *, #87078, .F. ) ;
#32593=AXIS2_PLACEMENT_3D ( 'NONE', #33822, #85505, #125432 ) ;
#32594=ORIENTED_EDGE ( 'NONE', *, *, #827, .T. ) ;
#32595=CARTESIAN_POINT ( 'NONE',  ( -3.150000000000029221, 12.50000000000000000, -1.883746621131363597 ) ) ;
#32596=DIRECTION ( 'NONE',  ( 0.000000000000000000, 0.000000000000000000, -1.000000000000000000 ) ) ;
#32597=EDGE_CURVE ( 'NONE', #61381, #40379, #111187, .T. ) ;
#32598=PLANE ( 'NONE',  #15267 ) ;
#32599=DIRECTION ( 'NONE',  ( 0.000000000000000000, 1.000000000000000000, 0.000000000000000000 ) ) ;
#32600=EDGE_CURVE ( 'NONE', #19176, #75526, #51659, .T. ) ;
#32601=EDGE_CURVE ( 'NONE', #115027, #109720, #60711, .T. ) ;
#32602=CARTESIAN_POINT ( 'NONE',  ( 6.899999999999926636, 12.50000000000000000, 0.3464101615137736845 ) ) ;
#32603=EDGE_CURVE ( 'NONE', #37202, #4262, #592, .T. ) ;
#32604=ORIENTED_EDGE ( 'NONE', *, *, #495, .F. ) ;
#32605=ORIENTED_EDGE ( 'NONE', *, *, #4064, .F. ) ;
#32606=DIRECTION ( 'NONE',  ( -0.000000000000000000, 1.000000000000000000, -0.000000000000000000 ) ) ;
#32607=CIRCLE ( 'NONE', #15838, 0.09999999999999999167 ) ;
#32608=CIRCLE ( 'NONE', #118252, 0.06509327318403745899 ) ;
#32609=CARTESIAN_POINT ( 'NONE',  ( 14.54999999999989235, 2.500000000000000000, -2.165063509461101710 ) ) ;
#32610=ADVANCED_FACE ( 'NONE', ( #33312 ), #123390, .T. ) ;
#32611=DIRECTION ( 'NONE',  ( -0.000000000000000000, -1.000000000000000000, -0.000000000000000000 ) ) ;
#32612=ORIENTED_EDGE ( 'NONE', *, *, #77399, .F. ) ;
#32613=VERTEX_POINT ( 'NONE', #83050 ) ;
#32614=ADVANCED_FACE ( 'NONE', ( #53587 ), #5738, .T. ) ;
#32615=PLANE ( 'NONE',  #20626 ) ;
#32616=ORIENTED_EDGE ( 'NONE', *, *, #105912, .F. ) ;
#32617=DIRECTION ( 'NONE',  ( 0.000000000000000000, 0.000000000000000000, -1.000000000000000000 ) ) ;
#32618=DIRECTION ( 'NONE',  ( -0.000000000000000000, 1.000000000000000000, -0.000000000000000000 ) ) ;
#32619=EDGE_CURVE ( 'NONE', #107723, #67419, #29316, .T. ) ;
#32620=EDGE_CURVE ( 'NONE', #70966, #119822, #74505, .T. ) ;
#32621=DIRECTION ( 'NONE',  ( 0.000000000000000000, 0.000000000000000000, 1.000000000000000000 ) ) ;
#32622=ORIENTED_EDGE ( 'NONE', *, *, #124056, .T. ) ;
#32623=DIRECTION ( 'NONE',  ( -0.000000000000000000, 1.000000000000000000, -0.000000000000000000 ) ) ;
#32624=CARTESIAN_POINT ( 'NONE',  ( 6.249999999999968914, 2.500000000000000000, -6.495190528383302464 ) ) ;
#32625=DIRECTION ( 'NONE',  ( 0.000000000000000000, 0.000000000000000000, 1.000000000000000000 ) ) ;
#32626=DIRECTION ( 'NONE',  ( 0.000000000000000000, 0.000000000000000000, 1.000000000000000000 ) ) ;
#32627=DIRECTION ( 'NONE',  ( 0.000000000000000000, 1.000000000000000000, 0.000000000000000000 ) ) ;
#32628=ADVANCED_FACE ( 'NONE', ( #115050 ), #6294, .T. ) ;
#32629=ORIENTED_EDGE ( 'NONE', *, *, #17755, .T. ) ;
#32630=DIRECTION ( 'NONE',  ( 0.000000000000000000, 0.000000000000000000, 1.000000000000000000 ) ) ;
#32631=AXIS2_PLACEMENT_3D ( 'NONE', #112236, #102417, #123971 ) ;
#32632=VECTOR ( 'NONE', #112000, 1000.000000000000000 ) ;
#32633=DIRECTION ( 'NONE',  ( 0.000000000000000000, -0.000000000000000000, 1.000000000000000000 ) ) ;
#32634=ORIENTED_EDGE ( 'NONE', *, *, #1655, .T. ) ;
#32636=ORIENTED_EDGE ( 'NONE', *, *, #79007, .T. ) ;
#32638=LINE ( 'NONE', #72540, #44873 ) ;
#32639=DIRECTION ( 'NONE',  ( 0.000000000000000000, 0.000000000000000000, -1.000000000000000000 ) ) ;
#32640=DIRECTION ( 'NONE',  ( 0.000000000000000000, 0.000000000000000000, 1.000000000000000000 ) ) ;
#32641=DIRECTION ( 'NONE',  ( -0.000000000000000000, 1.000000000000000000, -0.000000000000000000 ) ) ;
#32642=DIRECTION ( 'NONE',  ( 0.000000000000000000, 1.000000000000000000, 0.000000000000000000 ) ) ;
#32643=FACE_OUTER_BOUND ( 'NONE', #9997, .T. ) ;
#32644=DIRECTION ( 'NONE',  ( -0.000000000000000000, -1.000000000000000000, -0.000000000000000000 ) ) ;
#32645=DIRECTION ( 'NONE',  ( -0.000000000000000000, -1.000000000000000000, -0.000000000000000000 ) ) ;
#32646=CONICAL_SURFACE ( 'NONE', #122416, 0.1000000000000002554, 0.003490658503988666988 ) ;
#32647=VERTEX_POINT ( 'NONE', #75780 ) ;
#32648=ORIENTED_EDGE ( 'NONE', *, *, #58897, .F. ) ;
#32649=AXIS2_PLACEMENT_3D ( 'NONE', #109362, #19704, #51109 ) ;
#32650=ORIENTED_EDGE ( 'NONE', *, *, #29137, .F. ) ;
#32651=VECTOR ( 'NONE', #60174, 1000.000000000000000 ) ;
#32652=EDGE_LOOP ( 'NONE', ( #12928, #101811, #92519, #48184 ) ) ;
#32653=CARTESIAN_POINT ( 'NONE',  ( 8.349999999999923261, 2.500000000000000000, 2.857883832488649301 ) ) ;
#32654=DIRECTION ( 'NONE',  ( -0.000000000000000000, 1.000000000000000000, -0.000000000000000000 ) ) ;
#32656=CARTESIAN_POINT ( 'NONE',  ( 7.899999999999924860, 2.500000000000000000, -4.230127018922201998 ) ) ;
#32657=ADVANCED_FACE ( 'NONE', ( #13637 ), #89939, .T. ) ;
#32658=EDGE_CURVE ( 'NONE', #87021, #128668, #54846, .T. ) ;
#32659=DIRECTION ( 'NONE',  ( 0.000000000000000000, 1.000000000000000000, 0.000000000000000000 ) ) ;
#32660=DIRECTION ( 'NONE',  ( -4.274815082592931898E-19, -0.9999939076577903929, -0.003490651415223739937 ) ) ;
#32661=ORIENTED_EDGE ( 'NONE', *, *, #32359, .T. ) ;
#32662=DIRECTION ( 'NONE',  ( 0.000000000000000000, -0.9999939076577903929, 0.003490651415223739937 ) ) ;
#32663=CIRCLE ( 'NONE', #59939, 0.06509327318403745899 ) ;
#32665=VERTEX_POINT ( 'NONE', #122965 ) ;
#32666=EDGE_LOOP ( 'NONE', ( #14152, #84076 ) ) ;
#32667=ORIENTED_EDGE ( 'NONE', *, *, #47230, .F. ) ;
#32668=ORIENTED_EDGE ( 'NONE', *, *, #31858, .F. ) ;
#32669=DIRECTION ( 'NONE',  ( -0.000000000000000000, 1.000000000000000000, -0.000000000000000000 ) ) ;
#32670=CIRCLE ( 'NONE', #101694, 0.06509327318403745899 ) ;
#32671=AXIS2_PLACEMENT_3D ( 'NONE', #25758, #17191, #75491 ) ;
#32672=CARTESIAN_POINT ( 'NONE',  ( 6.649999999999930189, 2.500000000000000000, 7.088010851410848190 ) ) ;
#32673=LINE ( 'NONE', #100723, #42024 ) ;
#32675=CARTESIAN_POINT ( 'NONE',  ( 12.69999999999990159, 2.500000000000000000, 4.576537180435972019 ) ) ;
#32676=ORIENTED_EDGE ( 'NONE', *, *, #76052, .F. ) ;
#32677=CONICAL_SURFACE ( 'NONE', #66087, 0.1000000000000002554, 0.003490658503988666988 ) ;
#32678=CARTESIAN_POINT ( 'NONE',  ( -10.65000000000000391, 2.500000000000000000, -2.411473670974874306 ) ) ;
#32679=ORIENTED_EDGE ( 'NONE', *, *, #98084, .T. ) ;
#32681=CARTESIAN_POINT ( 'NONE',  ( 2.500000000000002220, -1.499999999999999556, -9.999999999999998224 ) ) ;
#32682=LINE ( 'NONE', #62767, #6612 ) ;
#32683=DIRECTION ( 'NONE',  ( 0.000000000000000000, 1.000000000000000000, 0.000000000000000000 ) ) ;
#32684=CONICAL_SURFACE ( 'NONE', #61916, 0.09999999999999982514, 0.003490658503988666988 ) ;
#32685=ORIENTED_EDGE ( 'NONE', *, *, #104918, .F. ) ;
#32687=VECTOR ( 'NONE', #52502, 1000.000000000000000 ) ;
#32688=EDGE_LOOP ( 'NONE', ( #73037, #35076 ) ) ;
#32689=ORIENTED_EDGE ( 'NONE', *, *, #10125, .T. ) ;
#32690=DIRECTION ( 'NONE',  ( 0.000000000000000000, -0.9999939076577903929, 0.003490651415223739937 ) ) ;
#32691=CARTESIAN_POINT ( 'NONE',  ( -12.04999999999999716, 12.50000000000000000, -2.099970236277060476 ) ) ;
#32692=CARTESIAN_POINT ( 'NONE',  ( -6.050000000000017586, 2.500000000000000000, 6.148780366869520009 ) ) ;
#32693=FACE_BOUND ( 'NONE', #88814, .T. ) ;
#32694=LINE ( 'NONE', #91584, #122546 ) ;
#32695=PLANE ( 'NONE',  #119748 ) ;
#32696=DIRECTION ( 'NONE',  ( 0.000000000000000000, 0.000000000000000000, -1.000000000000000000 ) ) ;
#32697=ADVANCED_FACE ( 'NONE', ( #124255 ), #94140, .T. ) ;
#32698=DIRECTION ( 'NONE',  ( 0.000000000000000000, 0.000000000000000000, 1.000000000000000000 ) ) ;
#32699=FACE_OUTER_BOUND ( 'NONE', #21877, .T. ) ;
#32700=CARTESIAN_POINT ( 'NONE',  ( 12.09999999999990195, 2.500000000000000000, -0.5928203230275541635 ) ) ;
#32701=ORIENTED_EDGE ( 'NONE', *, *, #84164, .T. ) ;
#32702=DIRECTION ( 'NONE',  ( -0.000000000000000000, -1.000000000000000000, -0.000000000000000000 ) ) ;
#32703=ORIENTED_EDGE ( 'NONE', *, *, #10091, .F. ) ;
#32704=ORIENTED_EDGE ( 'NONE', *, *, #88023, .F. ) ;
#32705=ADVANCED_FACE ( 'NONE', ( #114418 ), #87865, .T. ) ;
#32706=DIRECTION ( 'NONE',  ( -0.000000000000000000, 1.000000000000000000, -0.000000000000000000 ) ) ;
#32707=CARTESIAN_POINT ( 'NONE',  ( 5.599999999999934808, 2.500000000000000000, -3.983716857408426293 ) ) ;
#32708=EDGE_CURVE ( 'NONE', #102277, #124065, #23467, .T. ) ;
#32709=FACE_BOUND ( 'NONE', #47079, .T. ) ;
#32710=DIRECTION ( 'NONE',  ( -4.274815082592931898E-19, -0.9999939076577903929, -0.003490651415223739937 ) ) ;
#32711=CIRCLE ( 'NONE', #128858, 0.06509327318403745899 ) ;
#32712=CIRCLE ( 'NONE', #97519, 0.1000000000000002554 ) ;
#32713=ORIENTED_EDGE ( 'NONE', *, *, #47230, .T. ) ;
#32714=DIRECTION ( 'NONE',  ( 0.000000000000000000, 1.000000000000000000, 0.000000000000000000 ) ) ;
#32715=ADVANCED_FACE ( 'NONE', ( #64677 ), #98254, .T. ) ;
#32716=CARTESIAN_POINT ( 'NONE',  ( 9.349999999999916156, 12.50000000000000000, -1.818653347947326138 ) ) ;
#32717=EDGE_LOOP ( 'NONE', ( #61318, #8519 ) ) ;
#32718=FACE_OUTER_BOUND ( 'NONE', #47220, .T. ) ;
#32719=DIRECTION ( 'NONE',  ( -0.000000000000000000, 1.000000000000000000, -0.000000000000000000 ) ) ;
#32720=AXIS2_PLACEMENT_3D ( 'NONE', #4587, #94954, #114566 ) ;
#32721=AXIS2_PLACEMENT_3D ( 'NONE', #20126, #70504, #110429 ) ;
#32722=ORIENTED_EDGE ( 'NONE', *, *, #86460, .T. ) ;
#32723=DIRECTION ( 'NONE',  ( 0.000000000000000000, 0.000000000000000000, 1.000000000000000000 ) ) ;
#32724=DIRECTION ( 'NONE',  ( 0.000000000000000000, 1.000000000000000000, 0.000000000000000000 ) ) ;
#32726=CONICAL_SURFACE ( 'NONE', #41044, 0.1000000000000000472, 0.003490658503988666988 ) ;
#32727=ORIENTED_EDGE ( 'NONE', *, *, #44494, .F. ) ;
#32728=VECTOR ( 'NONE', #94232, 1000.000000000000000 ) ;
#32729=DIRECTION ( 'NONE',  ( 0.000000000000000000, 1.000000000000000000, 0.000000000000000000 ) ) ;
#32730=DIRECTION ( 'NONE',  ( 0.000000000000000000, 0.000000000000000000, -1.000000000000000000 ) ) ;
#32731=DIRECTION ( 'NONE',  ( -0.000000000000000000, 1.000000000000000000, -0.000000000000000000 ) ) ;
#32732=ORIENTED_EDGE ( 'NONE', *, *, #96914, .F. ) ;
#32733=ORIENTED_EDGE ( 'NONE', *, *, #43960, .T. ) ;
#32734=DIRECTION ( 'NONE',  ( 0.000000000000000000, 0.000000000000000000, 1.000000000000000000 ) ) ;
#32735=ORIENTED_EDGE ( 'NONE', *, *, #34224, .T. ) ;
#32736=DIRECTION ( 'NONE',  ( -0.000000000000000000, -1.000000000000000000, -0.000000000000000000 ) ) ;
#32737=DIRECTION ( 'NONE',  ( -0.000000000000000000, -1.000000000000000000, -0.000000000000000000 ) ) ;
#32738=EDGE_CURVE ( 'NONE', #87143, #28223, #25384, .T. ) ;
#32739=VERTEX_POINT ( 'NONE', #103327 ) ;
#32740=DIRECTION ( 'NONE',  ( 0.000000000000000000, 0.000000000000000000, -1.000000000000000000 ) ) ;
#32741=DIRECTION ( 'NONE',  ( 0.000000000000000000, 1.000000000000000000, 0.000000000000000000 ) ) ;
#32742=DIRECTION ( 'NONE',  ( 0.000000000000000000, 0.000000000000000000, -1.000000000000000000 ) ) ;
#32744=EDGE_CURVE ( 'NONE', #48591, #24755, #71161, .T. ) ;
#32745=CIRCLE ( 'NONE', #128898, 0.09999999999999982514 ) ;
#32746=DIRECTION ( 'NONE',  ( 0.000000000000000000, 1.000000000000000000, 0.000000000000000000 ) ) ;
#32747=EDGE_CURVE ( 'NONE', #76320, #115380, #15568, .T. ) ;
#32748=EDGE_LOOP ( 'NONE', ( #85854, #99184 ) ) ;
#32749=ORIENTED_EDGE ( 'NONE', *, *, #122118, .F. ) ;
#32750=CARTESIAN_POINT ( 'NONE',  ( -8.550000000000013145, 2.500000000000000000, -6.941600689897073906 ) ) ;
#32751=EDGE_LOOP ( 'NONE', ( #116325, #7610, #63660, #38853 ) ) ;
#32752=CIRCLE ( 'NONE', #34802, 0.09999999999999999167 ) ;
#32753=LINE ( 'NONE', #72664, #114126 ) ;
#32754=EDGE_CURVE ( 'NONE', #71951, #72177, #114970, .T. ) ;
#32755=EDGE_LOOP ( 'NONE', ( #110745, #52434 ) ) ;
#32756=EDGE_LOOP ( 'NONE', ( #28550, #27604, #6780, #1714 ) ) ;
#32757=EDGE_CURVE ( 'NONE', #29668, #34370, #104516, .T. ) ;
#32758=AXIS2_PLACEMENT_3D ( 'NONE', #80382, #51566, #109831 ) ;
#32759=EDGE_LOOP ( 'NONE', ( #58107, #12343 ) ) ;
#32760=ADVANCED_FACE ( 'NONE', ( #12981 ), #92870, .T. ) ;
#32761=FACE_OUTER_BOUND ( 'NONE', #69829, .T. ) ;
#32762=AXIS2_PLACEMENT_3D ( 'NONE', #104787, #68584, #106101 ) ;
#32763=CIRCLE ( 'NONE', #112258, 0.1000000000000002554 ) ;
#32764=CARTESIAN_POINT ( 'NONE',  ( -8.750000000000010658, 2.500000000000000000, -7.188010851410848723 ) ) ;
#32765=CARTESIAN_POINT ( 'NONE',  ( 6.849999999999927702, 12.50000000000000000, 2.511473670974873507 ) ) ;
#32766=AXIS2_PLACEMENT_3D ( 'NONE', #27010, #97030, #98306 ) ;
#32768=EDGE_CURVE ( 'NONE', #37336, #93396, #75270, .T. ) ;
#32769=CARTESIAN_POINT ( 'NONE',  ( -3.350000000000028511, 12.50000000000000000, 2.857883832488649301 ) ) ;
#32772=CARTESIAN_POINT ( 'NONE',  ( 4.999999999999935163, 12.50000000000000000, 3.572213422710607489 ) ) ;
#32773=DIRECTION ( 'NONE',  ( 0.000000000000000000, 0.000000000000000000, -1.000000000000000000 ) ) ;
#32774=CARTESIAN_POINT ( 'NONE',  ( -2.950000000000029932, 12.50000000000000000, 2.230156782645134950 ) ) ;
#32775=EDGE_CURVE ( 'NONE', #79205, #100057, #92004, .T. ) ;
#32776=AXIS2_PLACEMENT_3D ( 'NONE', #121511, #44092, #125238 ) ;
#32777=VERTEX_POINT ( 'NONE', #7677 ) ;
#32778=VECTOR ( 'NONE', #109185, 1000.000000000000000 ) ;
#32779=CIRCLE ( 'NONE', #74517, 0.1000000000000002554 ) ;
#32780=CARTESIAN_POINT ( 'NONE',  ( 0.3999999999999568345, 2.500000000000000000, -3.637306695894650055 ) ) ;
#32781=ORIENTED_EDGE ( 'NONE', *, *, #66742, .F. ) ;
#32782=ORIENTED_EDGE ( 'NONE', *, *, #98613, .F. ) ;
#32783=DIRECTION ( 'NONE',  ( -0.000000000000000000, 1.000000000000000000, -0.000000000000000000 ) ) ;
#32784=PLANE ( 'NONE',  #51851 ) ;
#32785=CARTESIAN_POINT ( 'NONE',  ( 10.79999999999991367, 2.500000000000000000, -2.385244779468109755E-15 ) ) ;
#32786=CARTESIAN_POINT ( 'NONE',  ( 8.349999999999919709, 2.500000000000000000, 6.395190528383296602 ) ) ;
#32787=FACE_OUTER_BOUND ( 'NONE', #13857, .T. ) ;
#32788=DIRECTION ( 'NONE',  ( 0.000000000000000000, 0.000000000000000000, 1.000000000000000000 ) ) ;
#32789=CARTESIAN_POINT ( 'NONE',  ( 9.799999999999915445, 2.500000000000000000, 3.883716857408421319 ) ) ;
#32790=VERTEX_POINT ( 'NONE', #87533 ) ;
#32791=VERTEX_POINT ( 'NONE', #16202 ) ;
#32792=VERTEX_POINT ( 'NONE', #57445 ) ;
#32793=VERTEX_POINT ( 'NONE', #96703 ) ;
#32794=ORIENTED_EDGE ( 'NONE', *, *, #2862, .F. ) ;
#32795=DIRECTION ( 'NONE',  ( 0.000000000000000000, 1.000000000000000000, 0.000000000000000000 ) ) ;
#32797=VECTOR ( 'NONE', #86481, 1000.000000000000000 ) ;
#32798=CARTESIAN_POINT ( 'NONE',  ( -7.300000000000013145, 2.500000000000000000, 3.883716857408420431 ) ) ;
#32799=EDGE_CURVE ( 'NONE', #121834, #121812, #108721, .T. ) ;
#32800=CIRCLE ( 'NONE', #112299, 0.1000000000000000472 ) ;
#32801=DIRECTION ( 'NONE',  ( 0.000000000000000000, 0.000000000000000000, -1.000000000000000000 ) ) ;
#32802=CARTESIAN_POINT ( 'NONE',  ( 87.50000000000001421, -1.433398978532512302, 7.395196794792774142 ) ) ;
#32803=EDGE_LOOP ( 'NONE', ( #53778, #81641, #121553, #80992 ) ) ;
#32804=DIRECTION ( 'NONE',  ( 0.000000000000000000, 0.000000000000000000, -1.000000000000000000 ) ) ;
#32805=CARTESIAN_POINT ( 'NONE',  ( 9.399999999999915090, 2.500000000000000000, 4.776537180435972196 ) ) ;
#32806=CARTESIAN_POINT ( 'NONE',  ( 3.349999999999945466, 12.50000000000000000, -2.099970236277064473 ) ) ;
#32807=CONICAL_SURFACE ( 'NONE', #128956, 0.09999999999999982514, 0.003490658503988666988 ) ;
#32808=AXIS2_PLACEMENT_3D ( 'NONE', #108814, #19133, #80671 ) ;
#32809=DIRECTION ( 'NONE',  ( -0.000000000000000000, 1.000000000000000000, -0.000000000000000000 ) ) ;
#32810=EDGE_CURVE ( 'NONE', #527, #15992, #37800, .T. ) ;
#32811=ORIENTED_EDGE ( 'NONE', *, *, #59637, .F. ) ;
#32812=ORIENTED_EDGE ( 'NONE', *, *, #15977, .F. ) ;
#32813=VERTEX_POINT ( 'NONE', #77707 ) ;
#32814=CARTESIAN_POINT ( 'NONE',  ( -11.24999999999996270, 12.50000000000000000, 6.495190528383297135 ) ) ;
#32815=CONICAL_SURFACE ( 'NONE', #85011, 0.1000000000000002554, 0.003490658503988666988 ) ;
#32816=CIRCLE ( 'NONE', #105951, 0.06509327318403745899 ) ;
#32817=CARTESIAN_POINT ( 'NONE',  ( -11.04999999999999893, 2.500000000000000000, 1.818653347947321475 ) ) ;
#32818=CARTESIAN_POINT ( 'NONE',  ( -4.800000000000022915, 2.500000000000000000, 3.983716857408420076 ) ) ;
#32819=CIRCLE ( 'NONE', #26540, 0.1000000000000002554 ) ;
#32820=VERTEX_POINT ( 'NONE', #118290 ) ;
#32821=LINE ( 'NONE', #112654, #78867 ) ;
#32822=FACE_OUTER_BOUND ( 'NONE', #8205, .T. ) ;
#32823=FACE_OUTER_BOUND ( 'NONE', #64444, .T. ) ;
#32824=CARTESIAN_POINT ( 'NONE',  ( -13.29999999999999005, 12.50000000000000000, -0.06509327318403558549 ) ) ;
#32825=CARTESIAN_POINT ( 'NONE',  ( 3.749999999999938716, 2.500000000000000000, 7.088010851410848190 ) ) ;
#32826=ORIENTED_EDGE ( 'NONE', *, *, #14298, .T. ) ;
#32827=VERTEX_POINT ( 'NONE', #67219 ) ;
#32828=DIRECTION ( 'NONE',  ( -0.000000000000000000, -1.000000000000000000, -0.000000000000000000 ) ) ;
#32829=CIRCLE ( 'NONE', #116421, 0.1000000000000000472 ) ;
#32830=DIRECTION ( 'NONE',  ( 0.000000000000000000, 1.000000000000000000, 0.000000000000000000 ) ) ;
#32831=AXIS2_PLACEMENT_3D ( 'NONE', #43850, #11126, #112578 ) ;
#32832=DIRECTION ( 'NONE',  ( 0.000000000000000000, 0.000000000000000000, 1.000000000000000000 ) ) ;
#32833=CIRCLE ( 'NONE', #110189, 0.06509327318403745899 ) ;
#32834=DIRECTION ( 'NONE',  ( 0.000000000000000000, 1.000000000000000000, 0.000000000000000000 ) ) ;
#32835=EDGE_CURVE ( 'NONE', #54227, #85597, #79582, .T. ) ;
#32836=ORIENTED_EDGE ( 'NONE', *, *, #57723, .F. ) ;
#32837=VECTOR ( 'NONE', #79365, 1000.000000000000000 ) ;
#32838=EDGE_LOOP ( 'NONE', ( #54253, #3812, #58106, #61435 ) ) ;
#32839=DIRECTION ( 'NONE',  ( 0.000000000000000000, 0.000000000000000000, 1.000000000000000000 ) ) ;
#32840=DIRECTION ( 'NONE',  ( 0.000000000000000000, 1.000000000000000000, 0.000000000000000000 ) ) ;
#32841=AXIS2_PLACEMENT_3D ( 'NONE', #2403, #43662, #84200 ) ;
#32842=CARTESIAN_POINT ( 'NONE',  ( -5.650000000000019895, 12.50000000000000000, 6.906693963081109722 ) ) ;
#32843=CONICAL_SURFACE ( 'NONE', #36949, 0.1000000000000000472, 0.003490658503988666988 ) ;
#32844=DIRECTION ( 'NONE',  ( -0.000000000000000000, 1.000000000000000000, -0.000000000000000000 ) ) ;
#32845=ORIENTED_EDGE ( 'NONE', *, *, #25165, .T. ) ;
#32846=EDGE_CURVE ( 'NONE', #4275, #53990, #102549, .T. ) ;
#32847=DIRECTION ( 'NONE',  ( 0.000000000000000000, 0.000000000000000000, 1.000000000000000000 ) ) ;
#32848=AXIS2_PLACEMENT_3D ( 'NONE', #52436, #20410, #92351 ) ;
#32849=DIRECTION ( 'NONE',  ( -0.000000000000000000, 1.000000000000000000, -0.000000000000000000 ) ) ;
#32850=VERTEX_POINT ( 'NONE', #107828 ) ;
#32851=EDGE_CURVE ( 'NONE', #59330, #34614, #123475, .T. ) ;
#32852=DIRECTION ( 'NONE',  ( -4.274815082592931898E-19, -0.9999939076577903929, -0.003490651415223739937 ) ) ;
#32853=AXIS2_PLACEMENT_3D ( 'NONE', #83760, #121740, #43857 ) ;
#32854=ADVANCED_FACE ( 'NONE', ( #18149 ), #39884, .T. ) ;
#32855=ORIENTED_EDGE ( 'NONE', *, *, #34163, .F. ) ;
#32856=VECTOR ( 'NONE', #113322, 1000.000000000000000 ) ;
#32857=CARTESIAN_POINT ( 'NONE',  ( 6.649999999999927525, 2.500000000000000000, 2.265063509461097357 ) ) ;
#32858=AXIS2_PLACEMENT_3D ( 'NONE', #82826, #23901, #121435 ) ;
#32859=CONICAL_SURFACE ( 'NONE', #9765, 0.1000000000000002554, 0.003490658503988666988 ) ;
#32860=VERTEX_POINT ( 'NONE', #17497 ) ;
#32861=DIRECTION ( 'NONE',  ( -0.000000000000000000, 1.000000000000000000, -0.000000000000000000 ) ) ;
#32862=CARTESIAN_POINT ( 'NONE',  ( 11.24999999999994493, 2.500000000000000000, -2.165063509461101710 ) ) ;
#32863=EDGE_CURVE ( 'NONE', #117732, #107019, #86235, .T. ) ;
#32864=EDGE_LOOP ( 'NONE', ( #14613, #4845 ) ) ;
#32865=ORIENTED_EDGE ( 'NONE', *, *, #24349, .F. ) ;
#32866=ADVANCED_FACE ( 'NONE', ( #88159 ), #56573, .T. ) ;
#32871=DIRECTION ( 'NONE',  ( 0.000000000000000000, 1.000000000000000000, 0.000000000000000000 ) ) ;
#32872=DIRECTION ( 'NONE',  ( 0.000000000000000000, 0.000000000000000000, 1.000000000000000000 ) ) ;
#32873=CARTESIAN_POINT ( 'NONE',  ( 4.199999999999941558, 2.500000000000000000, -4.230127018922201998 ) ) ;
#32874=DIRECTION ( 'NONE',  ( 0.000000000000000000, -0.9999939076577903929, 0.003490651415223739937 ) ) ;
#32875=DIRECTION ( 'NONE',  ( 0.000000000000000000, 0.000000000000000000, 1.000000000000000000 ) ) ;
#32876=AXIS2_PLACEMENT_3D ( 'NONE', #6932, #8243, #87445 ) ;
#32877=EDGE_LOOP ( 'NONE', ( #66824, #19876, #127185, #26777 ) ) ;
#32878=ORIENTED_EDGE ( 'NONE', *, *, #83839, .T. ) ;
#32879=DIRECTION ( 'NONE',  ( 0.000000000000000000, 0.000000000000000000, 1.000000000000000000 ) ) ;
#32880=EDGE_LOOP ( 'NONE', ( #31650, #57813, #18195, #25338 ) ) ;
#32881=CARTESIAN_POINT ( 'NONE',  ( 5.599999999999934808, 2.500000000000000000, -4.676537180435978769 ) ) ;
#32882=DIRECTION ( 'NONE',  ( 0.000000000000000000, 1.000000000000000000, 0.000000000000000000 ) ) ;
#32883=DIRECTION ( 'NONE',  ( 0.000000000000000000, -0.000000000000000000, 1.000000000000000000 ) ) ;
#32884=ORIENTED_EDGE ( 'NONE', *, *, #119762, .F. ) ;
#32885=ORIENTED_EDGE ( 'NONE', *, *, #89153, .T. ) ;
#32886=FACE_BOUND ( 'NONE', #62678, .T. ) ;
#32887=ORIENTED_EDGE ( 'NONE', *, *, #118594, .T. ) ;
#32888=CARTESIAN_POINT ( 'NONE',  ( -4.150000000000025224, 12.50000000000000000, 7.253104124594885960 ) ) ;
#32889=PLANE ( 'NONE',  #93748 ) ;
#32890=CARTESIAN_POINT ( 'NONE',  ( 8.299999999999922551, 2.500000000000000000, 4.230127018922196669 ) ) ;
#32891=LINE ( 'NONE', #91793, #82851 ) ;
#32892=AXIS2_PLACEMENT_3D ( 'NONE', #65393, #73938, #15638 ) ;
#32893=LINE ( 'NONE', #119966, #68071 ) ;
#32894=CIRCLE ( 'NONE', #57923, 0.06509327318403745899 ) ;
#32895=DIRECTION ( 'NONE',  ( 0.000000000000000000, 1.000000000000000000, 0.000000000000000000 ) ) ;
#32896=DIRECTION ( 'NONE',  ( -0.000000000000000000, 1.000000000000000000, -0.000000000000000000 ) ) ;
#32897=DIRECTION ( 'NONE',  ( 0.000000000000000000, 0.000000000000000000, 1.000000000000000000 ) ) ;
#32898=DIRECTION ( 'NONE',  ( 0.000000000000000000, 0.000000000000000000, 1.000000000000000000 ) ) ;
#32899=PLANE ( 'NONE',  #77699 ) ;
#32900=CARTESIAN_POINT ( 'NONE',  ( 4.799999999999937650, 2.500000000000000000, -3.983716857408426293 ) ) ;
#32901=AXIS2_PLACEMENT_3D ( 'NONE', #73858, #41843, #83686 ) ;
#32902=CONICAL_SURFACE ( 'NONE', #39168, 0.09999999999999999167, 0.003490658503988666988 ) ;
#32903=ADVANCED_FACE ( 'NONE', ( #76441 ), #26693, .T. ) ;
#32904=EDGE_LOOP ( 'NONE', ( #71241, #34992, #74017, #128775 ) ) ;
#32905=ORIENTED_EDGE ( 'NONE', *, *, #122973, .T. ) ;
#32906=ORIENTED_EDGE ( 'NONE', *, *, #6711, .F. ) ;
#32907=FACE_OUTER_BOUND ( 'NONE', #121237, .T. ) ;
#32908=EDGE_LOOP ( 'NONE', ( #48406, #100602 ) ) ;
#32909=ADVANCED_FACE ( 'NONE', ( #77083 ), #10590, .T. ) ;
#32910=LINE ( 'NONE', #85680, #92510 ) ;
#32911=ADVANCED_FACE ( 'NONE', ( #56767 ), #116983, .T. ) ;
#32912=EDGE_LOOP ( 'NONE', ( #51241, #34248, #81656, #107889 ) ) ;
#32913=ORIENTED_EDGE ( 'NONE', *, *, #76601, .F. ) ;
#32914=VERTEX_POINT ( 'NONE', #68538 ) ;
#32915=ADVANCED_FACE ( 'NONE', ( #108463 ), #18793, .T. ) ;
#32916=DIRECTION ( 'NONE',  ( 0.000000000000000000, 1.000000000000000000, 0.000000000000000000 ) ) ;
#32917=CIRCLE ( 'NONE', #20273, 0.1000000000000002554 ) ;
#32918=AXIS2_PLACEMENT_3D ( 'NONE', #85637, #44424, #5765 ) ;
#32919=EDGE_CURVE ( 'NONE', #112155, #18602, #8449, .T. ) ;
#32920=VECTOR ( 'NONE', #51234, 1000.000000000000000 ) ;
#32921=DIRECTION ( 'NONE',  ( 0.000000000000000000, 0.000000000000000000, 1.000000000000000000 ) ) ;
#32922=DIRECTION ( 'NONE',  ( 0.000000000000000000, 0.000000000000000000, 1.000000000000000000 ) ) ;
#32923=ADVANCED_FACE ( 'NONE', ( #1729 ), #50848, .T. ) ;
#32924=CARTESIAN_POINT ( 'NONE',  ( 48.83367117136233304, -2.320420702487481002, -5.300559035864880641 ) ) ;
#32925=DIRECTION ( 'NONE',  ( -4.274815082592931898E-19, -0.9999939076577903929, -0.003490651415223739937 ) ) ;
#32926=FACE_OUTER_BOUND ( 'NONE', #76301, .T. ) ;
#32927=VERTEX_POINT ( 'NONE', #50214 ) ;
#32928=FACE_OUTER_BOUND ( 'NONE', #8263, .T. ) ;
#32929=ADVANCED_FACE ( 'NONE', ( #90762 ), #29411, .T. ) ;
#32930=VERTEX_POINT ( 'NONE', #31218 ) ;
#32931=VECTOR ( 'NONE', #66345, 1000.000000000000000 ) ;
#32932=ADVANCED_FACE ( 'NONE', ( #1091 ), #115056, .T. ) ;
#32933=ORIENTED_EDGE ( 'NONE', *, *, #124967, .F. ) ;
#32934=ORIENTED_EDGE ( 'NONE', *, *, #13021, .T. ) ;
#32935=CARTESIAN_POINT ( 'NONE',  ( 5.199999999999935341, 12.50000000000000000, -0.2813168883297409439 ) ) ;
#32936=EDGE_LOOP ( 'NONE', ( #115576, #9405, #90209, #17371 ) ) ;
#32937=ORIENTED_EDGE ( 'NONE', *, *, #12471, .T. ) ;
#32938=ORIENTED_EDGE ( 'NONE', *, *, #109582, .T. ) ;
#32939=AXIS2_PLACEMENT_3D ( 'NONE', #77949, #72014, #60277 ) ;
#32941=DIRECTION ( 'NONE',  ( -0.000000000000000000, -1.000000000000000000, -0.000000000000000000 ) ) ;
#32942=DIRECTION ( 'NONE',  ( 0.000000000000000000, -0.9999939076577903929, 0.003490651415223739937 ) ) ;
#32943=DIRECTION ( 'NONE',  ( -0.000000000000000000, -1.000000000000000000, -0.000000000000000000 ) ) ;
#32944=LINE ( 'NONE', #82682, #79660 ) ;
#32945=VECTOR ( 'NONE', #88723, 1000.000000000000000 ) ;
#32946=DIRECTION ( 'NONE',  ( 0.000000000000000000, 0.000000000000000000, 1.000000000000000000 ) ) ;
#32947=VECTOR ( 'NONE', #66496, 1000.000000000000000 ) ;
#32948=ORIENTED_EDGE ( 'NONE', *, *, #104392, .F. ) ;
#32949=CIRCLE ( 'NONE', #26666, 0.06509327318403745899 ) ;
#32950=CARTESIAN_POINT ( 'NONE',  ( -1.450000000000035927, 2.500000000000000000, -6.148780366869526226 ) ) ;
#32951=VERTEX_POINT ( 'NONE', #9626 ) ;
#32952=FACE_OUTER_BOUND ( 'NONE', #33320, .T. ) ;
#32953=ORIENTED_EDGE ( 'NONE', *, *, #129238, .F. ) ;
#32954=FACE_OUTER_BOUND ( 'NONE', #33295, .T. ) ;
#32955=AXIS2_PLACEMENT_3D ( 'NONE', #49657, #117065, #68624 ) ;
#32956=EDGE_LOOP ( 'NONE', ( #125054, #71213 ) ) ;
#32957=CARTESIAN_POINT ( 'NONE',  ( 8.749999999999957367, 12.50000000000000000, 2.230156782645134950 ) ) ;
#32958=AXIS2_PLACEMENT_3D ( 'NONE', #75554, #55286, #55920 ) ;
#32959=CIRCLE ( 'NONE', #70486, 0.09999999999999982514 ) ;
#32960=CARTESIAN_POINT ( 'NONE',  ( -7.100000000000017408, 12.50000000000000000, 0.7579135962115869374 ) ) ;
#32962=EDGE_LOOP ( 'NONE', ( #93691, #37121 ) ) ;
#32963=DIRECTION ( 'NONE',  ( -0.000000000000000000, 1.000000000000000000, -0.000000000000000000 ) ) ;
#32964=CARTESIAN_POINT ( 'NONE',  ( 2.500000000000002220, 1.500000000000000444, -9.999999999999998224 ) ) ;
#32965=CARTESIAN_POINT ( 'NONE',  ( -9.600000000000006750, 2.500000000000000000, 3.637306695894644726 ) ) ;
#32966=CARTESIAN_POINT ( 'NONE',  ( -8.550000000000009592, 12.50000000000000000, 6.841600689897072485 ) ) ;
#32967=CARTESIAN_POINT ( 'NONE',  ( -3.750000000000025757, 12.50000000000000000, -2.922977105672691422 ) ) ;
#32969=EDGE_LOOP ( 'NONE', ( #53336, #125778 ) ) ;
#32970=CARTESIAN_POINT ( 'NONE',  ( 1.899999999999951283, 2.500000000000000000, -4.676537180435977881 ) ) ;
#32971=AXIS2_PLACEMENT_3D ( 'NONE', #86950, #14953, #126886 ) ;
#32972=ORIENTED_EDGE ( 'NONE', *, *, #26473, .F. ) ;
#32973=CARTESIAN_POINT ( 'NONE',  ( -6.450000000000017941, 12.50000000000000000, -2.511473670974877948 ) ) ;
#32974=DIRECTION ( 'NONE',  ( 0.000000000000000000, 0.000000000000000000, 1.000000000000000000 ) ) ;
#32976=LINE ( 'NONE', #91234, #15497 ) ;
#32977=CARTESIAN_POINT ( 'NONE',  ( 2.099999999999950351, 2.500000000000000000, -5.122947341949753763 ) ) ;
#32978=DIRECTION ( 'NONE',  ( -4.274815082592931898E-19, -0.9999939076577903929, -0.003490651415223739937 ) ) ;
#32979=DIRECTION ( 'NONE',  ( 0.000000000000000000, -0.000000000000000000, 1.000000000000000000 ) ) ;
#32980=ORIENTED_EDGE ( 'NONE', *, *, #116034, .F. ) ;
#32981=CIRCLE ( 'NONE', #64256, 0.06509327318403745899 ) ;
#32982=CARTESIAN_POINT ( 'NONE',  ( 7.099999999999928590, 12.50000000000000000, 4.330127018922196314 ) ) ;
#32983=AXIS2_PLACEMENT_3D ( 'NONE', #118757, #108922, #19253 ) ;
#32984=CARTESIAN_POINT ( 'NONE',  ( 2.499999999999947153, 2.500000000000000000, 3.537306695894645081 ) ) ;
#32985=CARTESIAN_POINT ( 'NONE',  ( 7.899999999999923084, 12.50000000000000000, -0.6277270498435167934 ) ) ;
#32986=EDGE_LOOP ( 'NONE', ( #8531, #129163, #44462, #26111 ) ) ;
#32987=AXIS2_PLACEMENT_3D ( 'NONE', #78815, #53047, #102146 ) ;
#32988=DIRECTION ( 'NONE',  ( 0.000000000000000000, 0.000000000000000000, -1.000000000000000000 ) ) ;
#32989=AXIS2_PLACEMENT_3D ( 'NONE', #94384, #15821, #55119 ) ;
#32990=AXIS2_PLACEMENT_3D ( 'NONE', #69343, #58264, #18315 ) ;
#32991=ORIENTED_EDGE ( 'NONE', *, *, #92988, .T. ) ;
#32992=EDGE_LOOP ( 'NONE', ( #54072, #28468 ) ) ;
#32993=DIRECTION ( 'NONE',  ( 0.000000000000000000, 1.000000000000000000, 0.000000000000000000 ) ) ;
#32994=ORIENTED_EDGE ( 'NONE', *, *, #17053, .F. ) ;
#32995=DIRECTION ( 'NONE',  ( 0.000000000000000000, 1.000000000000000000, 0.000000000000000000 ) ) ;
#32996=FACE_OUTER_BOUND ( 'NONE', #34471, .T. ) ;
#32997=DIRECTION ( 'NONE',  ( 0.000000000000000000, 0.000000000000000000, 1.000000000000000000 ) ) ;
#32998=ORIENTED_EDGE ( 'NONE', *, *, #38190, .T. ) ;
#32999=CIRCLE ( 'NONE', #122873, 0.1000000000000002554 ) ;
#33000=ADVANCED_FACE ( 'NONE', ( #129434 ), #109097, .T. ) ;
#33001=DIRECTION ( 'NONE',  ( 0.000000000000000000, 1.000000000000000000, 0.000000000000000000 ) ) ;
#33002=DIRECTION ( 'NONE',  ( 0.000000000000000000, 0.000000000000000000, 1.000000000000000000 ) ) ;
#33003=CIRCLE ( 'NONE', #76899, 0.09999999999999999167 ) ;
#33004=ADVANCED_FACE ( 'NONE', ( #10888 ), #132, .T. ) ;
#33005=EDGE_CURVE ( 'NONE', #4024, #88048, #16840, .T. ) ;
#33006=EDGE_LOOP ( 'NONE', ( #58878, #86698 ) ) ;
#33007=AXIS2_PLACEMENT_3D ( 'NONE', #110727, #121838, #21057 ) ;
#33009=EDGE_LOOP ( 'NONE', ( #122740, #48823, #95865, #108786 ) ) ;
#33010=VECTOR ( 'NONE', #42896, 1000.000000000000000 ) ;
#33011=PLANE ( 'NONE',  #79773 ) ;
#33012=CARTESIAN_POINT ( 'NONE',  ( 13.74999999999989697, 12.50000000000000000, 2.792790559304612064 ) ) ;
#33013=ADVANCED_FACE ( 'NONE', ( #31855 ), #58656, .T. ) ;
#33014=ADVANCED_FACE ( 'NONE', ( #101881 ), #30580, .T. ) ;
#33016=EDGE_CURVE ( 'NONE', #111375, #113182, #2196, .T. ) ;
#33017=ORIENTED_EDGE ( 'NONE', *, *, #62618, .F. ) ;
#33018=EDGE_CURVE ( 'NONE', #35370, #63286, #50332, .T. ) ;
#33019=CIRCLE ( 'NONE', #110267, 0.06509327318403745899 ) ;
#33020=PLANE ( 'NONE',  #46800 ) ;
#33022=EDGE_LOOP ( 'NONE', ( #91261, #125566 ) ) ;
#33023=DIRECTION ( 'NONE',  ( 0.000000000000000000, 1.000000000000000000, 0.000000000000000000 ) ) ;
#33024=DIRECTION ( 'NONE',  ( -0.000000000000000000, 1.000000000000000000, -0.000000000000000000 ) ) ;
#33025=AXIS2_PLACEMENT_3D ( 'NONE', #44732, #105575, #93822 ) ;
#33026=DIRECTION ( 'NONE',  ( 0.000000000000000000, 0.000000000000000000, 1.000000000000000000 ) ) ;
#33027=DIRECTION ( 'NONE',  ( 0.000000000000000000, 0.000000000000000000, 1.000000000000000000 ) ) ;
#33028=LINE ( 'NONE', #2237, #96828 ) ;
#33029=EDGE_CURVE ( 'NONE', #48343, #79731, #127684, .T. ) ;
#33030=DIRECTION ( 'NONE',  ( -0.000000000000000000, -1.000000000000000000, -0.000000000000000000 ) ) ;
#33031=AXIS2_PLACEMENT_3D ( 'NONE', #68925, #70871, #20487 ) ;
#33032=LINE ( 'NONE', #41561, #71271 ) ;
#33035=EDGE_LOOP ( 'NONE', ( #71128, #109016, #97990, #32629 ) ) ;
#33036=ORIENTED_EDGE ( 'NONE', *, *, #127719, .T. ) ;
#33037=ORIENTED_EDGE ( 'NONE', *, *, #98973, .T. ) ;
#33038=LINE ( 'NONE', #40269, #30766 ) ;
#33039=DIRECTION ( 'NONE',  ( 0.000000000000000000, -0.9999939076577903929, 0.003490651415223739937 ) ) ;
#33041=CIRCLE ( 'NONE', #62276, 0.09999999999999982514 ) ;
#33042=ORIENTED_EDGE ( 'NONE', *, *, #25035, .F. ) ;
#33043=FACE_BOUND ( 'NONE', #56914, .T. ) ;
#33044=FACE_OUTER_BOUND ( 'NONE', #116972, .T. ) ;
#33045=DIRECTION ( 'NONE',  ( -0.000000000000000000, 1.000000000000000000, -0.000000000000000000 ) ) ;
#33046=FACE_OUTER_BOUND ( 'NONE', #70472, .T. ) ;
#33047=CONICAL_SURFACE ( 'NONE', #74798, 0.1000000000000002554, 0.003490658503988666988 ) ;
#33048=CIRCLE ( 'NONE', #114489, 0.1000000000000002554 ) ;
#33049=CARTESIAN_POINT ( 'NONE',  ( -1.900000000000034994, 12.50000000000000000, -4.676537180435978769 ) ) ;
#33050=DIRECTION ( 'NONE',  ( 0.000000000000000000, 1.000000000000000000, 0.000000000000000000 ) ) ;
#33051=DIRECTION ( 'NONE',  ( 0.000000000000000000, 1.000000000000000000, 0.000000000000000000 ) ) ;
#33052=DIRECTION ( 'NONE',  ( 0.000000000000000000, 1.000000000000000000, 0.000000000000000000 ) ) ;
#33053=DIRECTION ( 'NONE',  ( 0.000000000000000000, 1.000000000000000000, 0.000000000000000000 ) ) ;
#33054=ADVANCED_FACE ( 'NONE', ( #431 ), #12188, .T. ) ;
#33055=DIRECTION ( 'NONE',  ( -0.000000000000000000, -1.000000000000000000, -0.000000000000000000 ) ) ;
#33056=EDGE_LOOP ( 'NONE', ( #26982, #15455 ) ) ;
#33057=EDGE_LOOP ( 'NONE', ( #20720, #64276, #69575, #22572 ) ) ;
#33058=ORIENTED_EDGE ( 'NONE', *, *, #18657, .T. ) ;
#33059=VERTEX_POINT ( 'NONE', #69174 ) ;
#33060=ORIENTED_EDGE ( 'NONE', *, *, #58136, .F. ) ;
#33061=ORIENTED_EDGE ( 'NONE', *, *, #84597, .F. ) ;
#33062=EDGE_CURVE ( 'NONE', #60396, #77451, #21069, .T. ) ;
#33063=DIRECTION ( 'NONE',  ( 0.000000000000000000, -0.9999939076577903929, 0.003490651415223739937 ) ) ;
#33064=EDGE_CURVE ( 'NONE', #59538, #890, #18919, .T. ) ;
#33065=ORIENTED_EDGE ( 'NONE', *, *, #18396, .F. ) ;
#33066=VERTEX_POINT ( 'NONE', #63240 ) ;
#33067=EDGE_CURVE ( 'NONE', #70330, #408, #119272, .T. ) ;
#33068=EDGE_CURVE ( 'NONE', #101913, #110045, #94238, .T. ) ;
#33069=CARTESIAN_POINT ( 'NONE',  ( 13.51931942374044660, -2.499999999999746869, 8.074217332244989720 ) ) ;
#33070=AXIS2_PLACEMENT_3D ( 'NONE', #100176, #109995, #79884 ) ;
#33071=CARTESIAN_POINT ( 'NONE',  ( 3.949999999999938005, 12.50000000000000000, 6.776507416713035248 ) ) ;
#33072=LINE ( 'NONE', #104365, #73962 ) ;
#33073=AXIS2_PLACEMENT_3D ( 'NONE', #31274, #41745, #122229 ) ;
#33074=ADVANCED_FACE ( 'NONE', ( #92703 ), #52386, .T. ) ;
#33075=EDGE_LOOP ( 'NONE', ( #122941, #108393, #85105, #52283 ) ) ;
#33076=DIRECTION ( 'NONE',  ( -0.000000000000000000, -1.000000000000000000, -0.000000000000000000 ) ) ;
#33077=EDGE_CURVE ( 'NONE', #79983, #37437, #34442, .T. ) ;
#33078=AXIS2_PLACEMENT_3D ( 'NONE', #24372, #64287, #64923 ) ;
#33079=ADVANCED_FACE ( 'NONE', ( #13479 ), #14785, .T. ) ;
#33080=ORIENTED_EDGE ( 'NONE', *, *, #7743, .F. ) ;
#33081=AXIS2_PLACEMENT_3D ( 'NONE', #50502, #41358, #90415 ) ;
#33082=EDGE_CURVE ( 'NONE', #15950, #79738, #69101, .T. ) ;
#33083=EDGE_LOOP ( 'NONE', ( #94896, #34733 ) ) ;
#33084=DIRECTION ( 'NONE',  ( 0.000000000000000000, 0.000000000000000000, 1.000000000000000000 ) ) ;
#33085=DIRECTION ( 'NONE',  ( -0.000000000000000000, 1.000000000000000000, -0.000000000000000000 ) ) ;
#33086=VERTEX_POINT ( 'NONE', #93989 ) ;
#33087=ADVANCED_FACE ( 'NONE', ( #93348 ), #32517, .T. ) ;
#33088=VECTOR ( 'NONE', #105916, 1000.000000000000000 ) ;
#33089=ORIENTED_EDGE ( 'NONE', *, *, #86931, .T. ) ;
#33090=DIRECTION ( 'NONE',  ( -0.000000000000000000, -1.000000000000000000, -0.000000000000000000 ) ) ;
#33091=AXIS2_PLACEMENT_3D ( 'NONE', #71281, #82426, #2012 ) ;
#33092=FACE_OUTER_BOUND ( 'NONE', #120097, .T. ) ;
#33093=DIRECTION ( 'NONE',  ( 0.000000000000000000, 1.000000000000000000, 0.000000000000000000 ) ) ;
#33094=CARTESIAN_POINT ( 'NONE',  ( -8.950000000000006395, 2.500000000000000000, 6.841600689897072485 ) ) ;
#33095=CARTESIAN_POINT ( 'NONE',  ( 7.899999999999923084, 12.50000000000000000, 0.6277270498435120194 ) ) ;
#33096=EDGE_LOOP ( 'NONE', ( #124831, #55410, #100557, #74610 ) ) ;
#33097=DIRECTION ( 'NONE',  ( -0.000000000000000000, 1.000000000000000000, -0.000000000000000000 ) ) ;
#33098=AXIS2_PLACEMENT_3D ( 'NONE', #70054, #20311, #129002 ) ;
#33099=VERTEX_POINT ( 'NONE', #102517 ) ;
#33100=CARTESIAN_POINT ( 'NONE',  ( 87.50000000000002842, 6.761363245278265488, 3.308765358479924146 ) ) ;
#33101=ORIENTED_EDGE ( 'NONE', *, *, #68302, .F. ) ;
#33102=LINE ( 'NONE', #23244, #83971 ) ;
#33103=FACE_OUTER_BOUND ( 'NONE', #33875, .T. ) ;
#33104=CIRCLE ( 'NONE', #28977, 0.06509327318403745899 ) ;
#33105=CARTESIAN_POINT ( 'NONE',  ( 2.949999999999945111, 12.50000000000000000, 2.165063509461097713 ) ) ;
#33106=DIRECTION ( 'NONE',  ( 0.000000000000000000, 0.000000000000000000, -1.000000000000000000 ) ) ;
#33107=ORIENTED_EDGE ( 'NONE', *, *, #101456, .T. ) ;
#33108=CARTESIAN_POINT ( 'NONE',  ( -5.850000000000021849, 2.500000000000000000, -7.088010851410853519 ) ) ;
#33109=AXIS2_PLACEMENT_3D ( 'NONE', #99434, #77831, #128905 ) ;
#33111=DIRECTION ( 'NONE',  ( 0.000000000000000000, -0.9999939076577903929, 0.003490651415223739937 ) ) ;
#33112=ORIENTED_EDGE ( 'NONE', *, *, #50466, .F. ) ;
#33113=ORIENTED_EDGE ( 'NONE', *, *, #125996, .T. ) ;
#33114=ORIENTED_EDGE ( 'NONE', *, *, #60573, .T. ) ;
#33115=DIRECTION ( 'NONE',  ( 0.000000000000000000, 0.000000000000000000, -1.000000000000000000 ) ) ;
#33116=DIRECTION ( 'NONE',  ( 0.000000000000000000, 1.000000000000000000, 0.000000000000000000 ) ) ;
#33118=FACE_OUTER_BOUND ( 'NONE', #59, .T. ) ;
#33119=PLANE ( 'NONE',  #40309 ) ;
#33120=FACE_OUTER_BOUND ( 'NONE', #86075, .T. ) ;
#33121=EDGE_CURVE ( 'NONE', #96527, #30923, #43618, .T. ) ;
#33122=CARTESIAN_POINT ( 'NONE',  ( 4.999999999999969802, 2.500000000000000000, 4.330127018922196314 ) ) ;
#33123=CARTESIAN_POINT ( 'NONE',  ( -8.300000000000011369, 2.500000000000000000, -2.276824562219559311E-15 ) ) ;
#33124=ORIENTED_EDGE ( 'NONE', *, *, #84490, .F. ) ;
#33125=DIRECTION ( 'NONE',  ( 0.000000000000000000, 0.000000000000000000, 1.000000000000000000 ) ) ;
#33126=ADVANCED_FACE ( 'NONE', ( #42987 ), #233, .T. ) ;
#33127=CARTESIAN_POINT ( 'NONE',  ( -5.600000000000020073, 2.500000000000000000, -0.2464101615137782308 ) ) ;
#33128=DIRECTION ( 'NONE',  ( 0.000000000000000000, -0.000000000000000000, 1.000000000000000000 ) ) ;
#33129=CARTESIAN_POINT ( 'NONE',  ( -5.650000000000023448, 2.500000000000000000, -6.148780366869526226 ) ) ;
#33130=ORIENTED_EDGE ( 'NONE', *, *, #113486, .F. ) ;
#33131=CARTESIAN_POINT ( 'NONE',  ( 4.549999999999935874, 2.500000000000000000, 6.495190528383297135 ) ) ;
#33132=CONICAL_SURFACE ( 'NONE', #43699, 0.09999999999999982514, 0.003490658503988666988 ) ;
#33133=DIRECTION ( 'NONE',  ( 0.000000000000000000, 0.000000000000000000, 1.000000000000000000 ) ) ;
#33134=DIRECTION ( 'NONE',  ( 0.000000000000000000, 0.000000000000000000, 1.000000000000000000 ) ) ;
#33135=ORIENTED_EDGE ( 'NONE', *, *, #94944, .F. ) ;
#33136=VERTEX_POINT ( 'NONE', #82893 ) ;
#33137=CARTESIAN_POINT ( 'NONE',  ( 13.09999999999990195, 2.500000000000000000, -4.676537180435978769 ) ) ;
#33138=ORIENTED_EDGE ( 'NONE', *, *, #92410, .F. ) ;
#33139=ORIENTED_EDGE ( 'NONE', *, *, #42241, .F. ) ;
#33140=CARTESIAN_POINT ( 'NONE',  ( -7.500000000000015099, 12.50000000000000000, -4.957854068765716882 ) ) ;
#33141=AXIS2_PLACEMENT_3D ( 'NONE', #17186, #97071, #111381 ) ;
#33142=ORIENTED_EDGE ( 'NONE', *, *, #123623, .F. ) ;
#33143=DIRECTION ( 'NONE',  ( 0.000000000000000000, -0.000000000000000000, 1.000000000000000000 ) ) ;
#33144=DIRECTION ( 'NONE',  ( -0.000000000000000000, -1.000000000000000000, -0.000000000000000000 ) ) ;
#33145=DIRECTION ( 'NONE',  ( 0.000000000000000000, 0.000000000000000000, 1.000000000000000000 ) ) ;
#33146=VERTEX_POINT ( 'NONE', #124089 ) ;
#33147=AXIS2_PLACEMENT_3D ( 'NONE', #19076, #119232, #120530 ) ;
#33148=EDGE_CURVE ( 'NONE', #7115, #31484, #83535, .T. ) ;
#33149=CIRCLE ( 'NONE', #64714, 0.1000000000000002554 ) ;
#33150=VECTOR ( 'NONE', #96629, 1000.000000000000000 ) ;
#33151=CARTESIAN_POINT ( 'NONE',  ( 8.549999999999918998, 2.500000000000000000, -1.718653347947326049 ) ) ;
#33152=DIRECTION ( 'NONE',  ( 0.000000000000000000, 1.000000000000000000, 0.000000000000000000 ) ) ;
#33153=ORIENTED_EDGE ( 'NONE', *, *, #97032, .F. ) ;
#33156=EDGE_CURVE ( 'NONE', #85507, #92060, #113631, .T. ) ;
#33157=CONICAL_SURFACE ( 'NONE', #81268, 0.1000000000000002554, 0.003490658503988666988 ) ;
#33158=ORIENTED_EDGE ( 'NONE', *, *, #119862, .F. ) ;
#33159=AXIS2_PLACEMENT_3D ( 'NONE', #51114, #1344, #1987 ) ;
#33160=AXIS2_PLACEMENT_3D ( 'NONE', #122906, #1823, #81679 ) ;
#33161=ORIENTED_EDGE ( 'NONE', *, *, #115815, .T. ) ;
#33162=ORIENTED_EDGE ( 'NONE', *, *, #81406, .T. ) ;
#33163=VERTEX_POINT ( 'NONE', #4287 ) ;
#33164=FACE_OUTER_BOUND ( 'NONE', #93605, .T. ) ;
#33165=CARTESIAN_POINT ( 'NONE',  ( 11.75764115780555485, 2.499999999999999556, 7.679135278102248385 ) ) ;
#33166=EDGE_CURVE ( 'NONE', #42431, #34783, #60878, .T. ) ;
#33167=EDGE_CURVE ( 'NONE', #3107, #67445, #94315, .T. ) ;
#33168=CARTESIAN_POINT ( 'NONE',  ( 9.999999999999912959, 12.50000000000000000, 3.637306695894644726 ) ) ;
#33169=EDGE_CURVE ( 'NONE', #45268, #111304, #52464, .T. ) ;
#33170=FACE_BOUND ( 'NONE', #87141, .T. ) ;
#33171=VERTEX_POINT ( 'NONE', #121947 ) ;
#33172=EDGE_CURVE ( 'NONE', #69112, #5314, #16930, .T. ) ;
#33174=EDGE_CURVE ( 'NONE', #116569, #113123, #35755, .T. ) ;
#33175=CONICAL_SURFACE ( 'NONE', #16502, 0.1000000000000000472, 0.003490658503988666988 ) ;
#33176=CARTESIAN_POINT ( 'NONE',  ( -8.550000000000011369, 12.50000000000000000, -2.576566944158915184 ) ) ;
#33177=DIRECTION ( 'NONE',  ( -4.274815082592931898E-19, -0.9999939076577903929, -0.003490651415223739937 ) ) ;
#33178=CARTESIAN_POINT ( 'NONE',  ( -13.29999999999999005, 12.50000000000000000, -4.395220292106237103 ) ) ;
#33179=CARTESIAN_POINT ( 'NONE',  ( 6.649999999999930189, 2.500000000000000000, -2.757883832488654097 ) ) ;
#33180=EDGE_CURVE ( 'NONE', #97627, #51148, #64981, .T. ) ;
#33181=DIRECTION ( 'NONE',  ( -0.000000000000000000, 1.000000000000000000, -0.000000000000000000 ) ) ;
#33182=ADVANCED_FACE ( 'NONE', ( #81392 ), #125621, .T. ) ;
#33183=AXIS2_PLACEMENT_3D ( 'NONE', #81012, #71181, #496 ) ;
#33185=PLANE ( 'NONE',  #93335 ) ;
#33186=ORIENTED_EDGE ( 'NONE', *, *, #1802, .T. ) ;
#33187=VERTEX_POINT ( 'NONE', #31636 ) ;
#33188=VERTEX_POINT ( 'NONE', #42101 ) ;
#33190=ORIENTED_EDGE ( 'NONE', *, *, #35216, .F. ) ;
#33191=ORIENTED_EDGE ( 'NONE', *, *, #77746, .T. ) ;
#33192=CIRCLE ( 'NONE', #6052, 0.06509327318403743123 ) ;
#33193=DIRECTION ( 'NONE',  ( 0.000000000000000000, -0.000000000000000000, 1.000000000000000000 ) ) ;
#33194=CARTESIAN_POINT ( 'NONE',  ( 15.83209681635554666, 2.500000000000000000, 5.404881881984142211 ) ) ;
#33195=ORIENTED_EDGE ( 'NONE', *, *, #11329, .F. ) ;
#33196=FACE_BOUND ( 'NONE', #36864, .T. ) ;
#33197=DIRECTION ( 'NONE',  ( -4.274815082592931898E-19, -0.9999939076577903929, -0.003490651415223739937 ) ) ;
#33198=CIRCLE ( 'NONE', #5967, 0.06509327318403745899 ) ;
#33200=VERTEX_POINT ( 'NONE', #82013 ) ;
#33201=DIRECTION ( 'NONE',  ( 0.000000000000000000, 0.000000000000000000, 1.000000000000000000 ) ) ;
#33202=DIRECTION ( 'NONE',  ( -0.000000000000000000, -1.000000000000000000, -0.000000000000000000 ) ) ;
#33203=DIRECTION ( 'NONE',  ( -0.000000000000000000, -1.000000000000000000, -0.000000000000000000 ) ) ;
#33204=EDGE_LOOP ( 'NONE', ( #128404, #82221 ) ) ;
#33205=CIRCLE ( 'NONE', #49930, 0.09999999999999982514 ) ;
#33206=DIRECTION ( 'NONE',  ( -0.000000000000000000, -1.000000000000000000, -0.000000000000000000 ) ) ;
#33207=CIRCLE ( 'NONE', #20676, 0.06509327318403745899 ) ;
#33208=ORIENTED_EDGE ( 'NONE', *, *, #29790, .F. ) ;
#33209=ORIENTED_EDGE ( 'NONE', *, *, #125068, .T. ) ;
#33210=ORIENTED_EDGE ( 'NONE', *, *, #1085, .F. ) ;
#33211=DIRECTION ( 'NONE',  ( 0.000000000000000000, 1.000000000000000000, 0.000000000000000000 ) ) ;
#33212=CARTESIAN_POINT ( 'NONE',  ( -8.950000000000008171, 2.500000000000000000, -2.411473670974877859 ) ) ;
#33213=DIRECTION ( 'NONE',  ( 0.000000000000000000, 0.000000000000000000, 1.000000000000000000 ) ) ;
#33214=CONICAL_SURFACE ( 'NONE', #118874, 0.09999999999999982514, 0.003490658503988666988 ) ;
#33215=ORIENTED_EDGE ( 'NONE', *, *, #83602, .T. ) ;
#33216=FACE_OUTER_BOUND ( 'NONE', #112621, .T. ) ;
#33217=CARTESIAN_POINT ( 'NONE',  ( -7.050000000000016698, 12.50000000000000000, -2.099970236277064473 ) ) ;
#33218=CIRCLE ( 'NONE', #3945, 0.06509327318403745899 ) ;
#33219=DIRECTION ( 'NONE',  ( 0.000000000000000000, 1.000000000000000000, 0.000000000000000000 ) ) ;
#33220=AXIS2_PLACEMENT_3D ( 'NONE', #102057, #109947, #110579 ) ;
#33222=ORIENTED_EDGE ( 'NONE', *, *, #65518, .T. ) ;
#33223=CIRCLE ( 'NONE', #91694, 0.06509327318403745899 ) ;
#33224=CARTESIAN_POINT ( 'NONE',  ( -4.600000000000028066, 12.50000000000000000, -5.022947341949754119 ) ) ;
#33225=ADVANCED_FACE ( 'NONE', ( #51926 ), #59834, .T. ) ;
#33226=EDGE_LOOP ( 'NONE', ( #9172, #109653, #69716, #103797 ) ) ;
#33228=ADVANCED_FACE ( 'NONE', ( #80743 ), #102640, .T. ) ;
#33229=CIRCLE ( 'NONE', #93759, 0.09999999999999982514 ) ;
#33230=EDGE_LOOP ( 'NONE', ( #14679, #90507 ) ) ;
#33231=ADVANCED_FACE ( 'NONE', ( #91844 ), #42010, .T. ) ;
#33232=ORIENTED_EDGE ( 'NONE', *, *, #81780, .T. ) ;
#33233=DIRECTION ( 'NONE',  ( 0.000000000000000000, 0.000000000000000000, 1.000000000000000000 ) ) ;
#33234=CARTESIAN_POINT ( 'NONE',  ( 14.59999999999989484, 2.500000000000000000, -0.6928203230275541413 ) ) ;
#33235=FACE_OUTER_BOUND ( 'NONE', #91347, .T. ) ;
#33236=CARTESIAN_POINT ( 'NONE',  ( 10.64999999999990976, 12.50000000000000000, 1.818653347947321475 ) ) ;
#33237=DIRECTION ( 'NONE',  ( 0.000000000000000000, 0.000000000000000000, 1.000000000000000000 ) ) ;
#33238=ORIENTED_EDGE ( 'NONE', *, *, #113676, .F. ) ;
#33239=ADVANCED_FACE ( 'NONE', ( #19885 ), #104772, .T. ) ;
#33240=EDGE_LOOP ( 'NONE', ( #118892, #51229, #37829, #36249 ) ) ;
#33241=CARTESIAN_POINT ( 'NONE',  ( -6.900000000000019007, 12.50000000000000000, -4.676537180435978769 ) ) ;
#33243=DIRECTION ( 'NONE',  ( 0.000000000000000000, 1.000000000000000000, 0.000000000000000000 ) ) ;
#33244=ORIENTED_EDGE ( 'NONE', *, *, #60280, .T. ) ;
#33245=VERTEX_POINT ( 'NONE', #122593 ) ;
#33246=DIRECTION ( 'NONE',  ( 0.000000000000000000, 0.000000000000000000, 1.000000000000000000 ) ) ;
#33247=ORIENTED_EDGE ( 'NONE', *, *, #44592, .F. ) ;
#33248=DIRECTION ( 'NONE',  ( 0.000000000000000000, -0.9999939076577903929, 0.003490651415223739937 ) ) ;
#33249=CARTESIAN_POINT ( 'NONE',  ( -0.4000000000000396572, 2.500000000000000000, 3.637306695894644726 ) ) ;
#33250=AXIS2_PLACEMENT_3D ( 'NONE', #47130, #74640, #46459 ) ;
#33251=CIRCLE ( 'NONE', #26875, 0.06509327318403745899 ) ;
#33252=FACE_OUTER_BOUND ( 'NONE', #117543, .T. ) ;
#33253=ORIENTED_EDGE ( 'NONE', *, *, #50577, .F. ) ;
#33254=CARTESIAN_POINT ( 'NONE',  ( -8.300000000000011369, 2.500000000000000000, -4.230127018922201998 ) ) ;
#33255=CARTESIAN_POINT ( 'NONE',  ( 0.000000000000000000, 2.500000000000000000, 0.000000000000000000 ) ) ;
#33256=DIRECTION ( 'NONE',  ( -0.000000000000000000, 1.000000000000000000, -0.000000000000000000 ) ) ;
#33257=CARTESIAN_POINT ( 'NONE',  ( 10.84999999999990905, 2.500000000000000000, 2.065063509461097624 ) ) ;
#33258=EDGE_CURVE ( 'NONE', #107723, #44898, #111470, .T. ) ;
#33259=CARTESIAN_POINT ( 'NONE',  ( 5.599999999999931255, 12.50000000000000000, 3.983716857408420076 ) ) ;
#33260=CIRCLE ( 'NONE', #18648, 0.06509327318403745899 ) ;
#33261=ORIENTED_EDGE ( 'NONE', *, *, #117831, .T. ) ;
#33262=VECTOR ( 'NONE', #128231, 1000.000000000000000 ) ;
#33263=AXIS2_PLACEMENT_3D ( 'NONE', #84569, #56384, #7927 ) ;
#33264=DIRECTION ( 'NONE',  ( 0.000000000000000000, 0.000000000000000000, 1.000000000000000000 ) ) ;
#33265=CARTESIAN_POINT ( 'NONE',  ( 65.40459994265785326, -3.824478557808927093, 5.306485876512247124 ) ) ;
#33266=ORIENTED_EDGE ( 'NONE', *, *, #64884, .T. ) ;
#33267=EDGE_LOOP ( 'NONE', ( #95076, #66238 ) ) ;
#33269=DIRECTION ( 'NONE',  ( 0.000000000000000000, 0.000000000000000000, 1.000000000000000000 ) ) ;
#33270=DIRECTION ( 'NONE',  ( 0.000000000000000000, 0.000000000000000000, -1.000000000000000000 ) ) ;
#33271=CIRCLE ( 'NONE', #114803, 0.09999999999999999167 ) ;
#33272=DIRECTION ( 'NONE',  ( 0.000000000000000000, -0.9999939076577903929, 0.003490651415223739937 ) ) ;
#33273=LINE ( 'NONE', #73807, #8795 ) ;
#33274=AXIS2_PLACEMENT_3D ( 'NONE', #17632, #79164, #97493 ) ;
#33275=CARTESIAN_POINT ( 'NONE',  ( 9.599999999999917932, 2.500000000000000000, 0.5928203230275495006 ) ) ;
#33276=DIRECTION ( 'NONE',  ( 0.000000000000000000, 0.000000000000000000, -1.000000000000000000 ) ) ;
#33277=ADVANCED_FACE ( 'NONE', ( #92479 ), #10685, .T. ) ;
#33278=CARTESIAN_POINT ( 'NONE',  ( -2.950000000000033484, 2.500000000000000000, -6.395190528383301931 ) ) ;
#33281=CIRCLE ( 'NONE', #39554, 0.06509327318403745899 ) ;
#33282=ORIENTED_EDGE ( 'NONE', *, *, #123460, .T. ) ;
#33283=ORIENTED_EDGE ( 'NONE', *, *, #118180, .T. ) ;
#33285=CIRCLE ( 'NONE', #112687, 0.06509327318403745899 ) ;
#33286=ORIENTED_EDGE ( 'NONE', *, *, #56487, .F. ) ;
#33287=ADVANCED_FACE ( 'NONE', ( #21825 ), #46211, .T. ) ;
#33288=DIRECTION ( 'NONE',  ( 0.000000000000000000, 1.000000000000000000, 0.000000000000000000 ) ) ;
#33289=DIRECTION ( 'NONE',  ( 0.000000000000000000, 0.000000000000000000, -1.000000000000000000 ) ) ;
#33290=ORIENTED_EDGE ( 'NONE', *, *, #114840, .F. ) ;
#33291=CARTESIAN_POINT ( 'NONE',  ( 7.099999999999925926, 12.50000000000000000, 0.6928203230275494784 ) ) ;
#33292=CIRCLE ( 'NONE', #106423, 0.06509327318403745899 ) ;
#33293=CARTESIAN_POINT ( 'NONE',  ( 3.349999999999942801, 2.500000000000000000, 2.857883832488649301 ) ) ;
#33294=CARTESIAN_POINT ( 'NONE',  ( -12.04999999999999716, 12.50000000000000000, -6.495190528383298911 ) ) ;
#33295=EDGE_LOOP ( 'NONE', ( #28055, #128522 ) ) ;
#33296=CARTESIAN_POINT ( 'NONE',  ( 15.39999999999989200, 2.500000000000000000, 0.6928203230275494784 ) ) ;
#33297=PLANE ( 'NONE',  #91813 ) ;
#33299=AXIS2_PLACEMENT_3D ( 'NONE', #95283, #46175, #84157 ) ;
#33300=EDGE_LOOP ( 'NONE', ( #6787, #25094 ) ) ;
#33301=ORIENTED_EDGE ( 'NONE', *, *, #30077, .F. ) ;
#33302=ORIENTED_EDGE ( 'NONE', *, *, #55346, .F. ) ;
#33303=DIRECTION ( 'NONE',  ( -4.274815082592931898E-19, -0.9999939076577903929, -0.003490651415223739937 ) ) ;
#33304=CIRCLE ( 'NONE', #106440, 0.09999999999999999167 ) ;
#33305=DIRECTION ( 'NONE',  ( -4.274815082592931898E-19, -0.9999939076577903929, -0.003490651415223739937 ) ) ;
#33306=DIRECTION ( 'NONE',  ( 0.000000000000000000, 1.000000000000000000, 0.000000000000000000 ) ) ;
#33307=CARTESIAN_POINT ( 'NONE',  ( 2.099999999999950351, 12.50000000000000000, -4.330127018922201643 ) ) ;
#33308=VERTEX_POINT ( 'NONE', #42770 ) ;
#33309=EDGE_CURVE ( 'NONE', #79506, #25742, #32944, .T. ) ;
#33310=CIRCLE ( 'NONE', #85604, 0.09999999999999982514 ) ;
#33311=AXIS2_PLACEMENT_3D ( 'NONE', #120259, #30599, #41070 ) ;
#33312=FACE_OUTER_BOUND ( 'NONE', #32522, .T. ) ;
#33313=VERTEX_POINT ( 'NONE', #60472 ) ;
#33315=CARTESIAN_POINT ( 'NONE',  ( 8.497934422629066731, -2.500000000000762057, -9.526046681109040293 ) ) ;
#33316=AXIS2_PLACEMENT_3D ( 'NONE', #115583, #25941, #106422 ) ;
#33317=DIRECTION ( 'NONE',  ( -4.274815082592931898E-19, -0.9999939076577903929, -0.003490651415223739937 ) ) ;
#33318=DIRECTION ( 'NONE',  ( -0.000000000000000000, 1.000000000000000000, -0.000000000000000000 ) ) ;
#33319=EDGE_CURVE ( 'NONE', #82277, #28259, #100374, .T. ) ;
#33320=EDGE_LOOP ( 'NONE', ( #104265, #121178, #101241, #42370 ) ) ;
#33321=AXIS2_PLACEMENT_3D ( 'NONE', #93345, #112978, #54061 ) ;
#33322=ORIENTED_EDGE ( 'NONE', *, *, #39887, .T. ) ;
#33323=ORIENTED_EDGE ( 'NONE', *, *, #86622, .T. ) ;
#33324=FACE_OUTER_BOUND ( 'NONE', #3761, .T. ) ;
#33325=DIRECTION ( 'NONE',  ( -0.000000000000000000, 1.000000000000000000, -0.000000000000000000 ) ) ;
#33326=EDGE_CURVE ( 'NONE', #117920, #69856, #110823, .T. ) ;
#33327=ADVANCED_FACE ( 'NONE', ( #96215 ), #65067, .T. ) ;
#33328=LINE ( 'NONE', #111872, #92022 ) ;
#33329=EDGE_CURVE ( 'NONE', #79083, #12477, #75451, .T. ) ;
#33330=FACE_BOUND ( 'NONE', #75332, .T. ) ;
#33331=ADVANCED_FACE ( 'NONE', ( #114570 ), #54608, .T. ) ;
#33332=DIRECTION ( 'NONE',  ( -0.000000000000000000, -1.000000000000000000, -0.000000000000000000 ) ) ;
#33333=LINE ( 'NONE', #73237, #71734 ) ;
#33334=LINE ( 'NONE', #44416, #1887 ) ;
#33336=CIRCLE ( 'NONE', #104416, 0.1000000000000000472 ) ;
#33338=ADVANCED_FACE ( 'NONE', ( #17663 ), #6521, .T. ) ;
#33339=DIRECTION ( 'NONE',  ( 0.000000000000000000, 0.000000000000000000, 1.000000000000000000 ) ) ;
#33340=ADVANCED_FACE ( 'NONE', ( #16983 ), #25537, .T. ) ;
#33341=FACE_OUTER_BOUND ( 'NONE', #108887, .T. ) ;
#33343=ADVANCED_FACE ( 'NONE', ( #124410 ), #92176, .T. ) ;
#33344=AXIS2_PLACEMENT_3D ( 'NONE', #35228, #124241, #26038 ) ;
#33345=EDGE_CURVE ( 'NONE', #50751, #65093, #86399, .T. ) ;
#33346=AXIS2_PLACEMENT_3D ( 'NONE', #18274, #66723, #9752 ) ;
#33347=DIRECTION ( 'NONE',  ( 0.000000000000000000, 0.000000000000000000, 1.000000000000000000 ) ) ;
#33348=ORIENTED_EDGE ( 'NONE', *, *, #120975, .T. ) ;
#33349=ORIENTED_EDGE ( 'NONE', *, *, #73254, .T. ) ;
#33350=DIRECTION ( 'NONE',  ( -0.000000000000000000, 1.000000000000000000, -0.000000000000000000 ) ) ;
#33351=FACE_BOUND ( 'NONE', #102293, .T. ) ;
#33352=EDGE_CURVE ( 'NONE', #110270, #57844, #126345, .T. ) ;
#33353=DIRECTION ( 'NONE',  ( -0.000000000000000000, -1.000000000000000000, -0.000000000000000000 ) ) ;
#33354=CIRCLE ( 'NONE', #64713, 0.06509327318403745899 ) ;
#33355=AXIS2_PLACEMENT_3D ( 'NONE', #124196, #85552, #84257 ) ;
#33356=CONICAL_SURFACE ( 'NONE', #58391, 0.1000000000000002554, 0.003490658503988666988 ) ;
#33357=EDGE_LOOP ( 'NONE', ( #89369, #53830, #72467, #50305 ) ) ;
#33358=CARTESIAN_POINT ( 'NONE',  ( 32.27111852103329426, 3.178312372602895675, 3.140919221358756452 ) ) ;
#33359=CARTESIAN_POINT ( 'NONE',  ( -3.300000000000027800, 2.500000000000000000, -2.276824562219559311E-15 ) ) ;
#33360=AXIS2_PLACEMENT_3D ( 'NONE', #73546, #63747, #13980 ) ;
#33361=ORIENTED_EDGE ( 'NONE', *, *, #106189, .T. ) ;
#33362=CARTESIAN_POINT ( 'NONE',  ( -3.350000000000031619, 2.500000000000000000, -7.288010851410854585 ) ) ;
#33363=DIRECTION ( 'NONE',  ( 0.000000000000000000, 1.000000000000000000, 0.000000000000000000 ) ) ;
#33364=CONICAL_SURFACE ( 'NONE', #127440, 0.1000000000000002554, 0.003490658503988666988 ) ;
#33365=VECTOR ( 'NONE', #81908, 1000.000000000000000 ) ;
#33366=ORIENTED_EDGE ( 'NONE', *, *, #41248, .F. ) ;
#33367=DIRECTION ( 'NONE',  ( 0.000000000000000000, 0.000000000000000000, -1.000000000000000000 ) ) ;
#33368=DIRECTION ( 'NONE',  ( 0.000000000000000000, 1.000000000000000000, 0.000000000000000000 ) ) ;
#33369=EDGE_LOOP ( 'NONE', ( #97393, #51488, #119364, #118651 ) ) ;
#33370=DIRECTION ( 'NONE',  ( 0.000000000000000000, 0.000000000000000000, -1.000000000000000000 ) ) ;
#33371=DIRECTION ( 'NONE',  ( 0.000000000000000000, 0.000000000000000000, 1.000000000000000000 ) ) ;
#33372=LINE ( 'NONE', #62184, #51433 ) ;
#33373=AXIS2_PLACEMENT_3D ( 'NONE', #63651, #52530, #64277 ) ;
#33374=EDGE_LOOP ( 'NONE', ( #90004, #73121 ) ) ;
#33376=DIRECTION ( 'NONE',  ( 0.000000000000000000, 1.000000000000000000, 0.000000000000000000 ) ) ;
#33377=EDGE_LOOP ( 'NONE', ( #111135, #92115, #80805, #78888 ) ) ;
#33378=CARTESIAN_POINT ( 'NONE',  ( -14.99999999999998224, 2.500000000000000000, -0.7928203230275518987 ) ) ;
#33379=DIRECTION ( 'NONE',  ( 0.000000000000000000, -0.000000000000000000, 1.000000000000000000 ) ) ;
#33380=EDGE_CURVE ( 'NONE', #102542, #84188, #39962, .T. ) ;
#33381=ORIENTED_EDGE ( 'NONE', *, *, #86315, .F. ) ;
#33382=CARTESIAN_POINT ( 'NONE',  ( -11.05000000000000071, 2.500000000000000000, -2.511473670974873951 ) ) ;
#33383=ADVANCED_FACE ( 'NONE', ( #85756 ), #10768, .T. ) ;
#33384=DIRECTION ( 'NONE',  ( 0.000000000000000000, -0.9999939076577903929, 0.003490651415223739937 ) ) ;
#33385=CARTESIAN_POINT ( 'NONE',  ( -7.900000000000014566, 2.500000000000000000, -3.737306695894649700 ) ) ;
#33387=FACE_OUTER_BOUND ( 'NONE', #75626, .T. ) ;
#33388=CARTESIAN_POINT ( 'NONE',  ( 2.499999999999981792, 12.50000000000000000, 4.330127018922196314 ) ) ;
#33389=EDGE_CURVE ( 'NONE', #110247, #16833, #47142, .T. ) ;
#33390=VERTEX_POINT ( 'NONE', #87046 ) ;
#33391=ORIENTED_EDGE ( 'NONE', *, *, #103819, .T. ) ;
#33392=CARTESIAN_POINT ( 'NONE',  ( -0.6500000000000403233, 12.50000000000000000, 6.213873640053558134 ) ) ;
#33393=ORIENTED_EDGE ( 'NONE', *, *, #60748, .F. ) ;
#33395=ORIENTED_EDGE ( 'NONE', *, *, #120350, .T. ) ;
#33396=ORIENTED_EDGE ( 'NONE', *, *, #121136, .F. ) ;
#33397=ORIENTED_EDGE ( 'NONE', *, *, #29686, .T. ) ;
#33398=AXIS2_PLACEMENT_3D ( 'NONE', #76848, #116751, #7441 ) ;
#33399=DIRECTION ( 'NONE',  ( 0.000000000000000000, 1.000000000000000000, 0.000000000000000000 ) ) ;
#33400=DIRECTION ( 'NONE',  ( -0.000000000000000000, 1.000000000000000000, -0.000000000000000000 ) ) ;
#33401=CARTESIAN_POINT ( 'NONE',  ( 12.29999999999990479, 12.50000000000000000, -3.983716857408426293 ) ) ;
#33403=AXIS2_PLACEMENT_3D ( 'NONE', #125355, #45523, #83515 ) ;
#33404=AXIS2_PLACEMENT_3D ( 'NONE', #52790, #107028, #15425 ) ;
#33405=DIRECTION ( 'NONE',  ( -0.000000000000000000, -1.000000000000000000, -0.000000000000000000 ) ) ;
#33406=DIRECTION ( 'NONE',  ( 0.000000000000000000, 0.000000000000000000, 1.000000000000000000 ) ) ;
#33407=FACE_OUTER_BOUND ( 'NONE', #5592, .T. ) ;
#33408=DIRECTION ( 'NONE',  ( 0.000000000000000000, 0.000000000000000000, 1.000000000000000000 ) ) ;
#33409=CARTESIAN_POINT ( 'NONE',  ( 1.049999999999954969, 2.500000000000000000, -6.741600689897077281 ) ) ;
#33410=AXIS2_PLACEMENT_3D ( 'NONE', #84696, #52653, #92590 ) ;
#33411=PLANE ( 'NONE',  #58206 ) ;
#33412=CIRCLE ( 'NONE', #106541, 0.06509327318403745899 ) ;
#33413=AXIS2_PLACEMENT_3D ( 'NONE', #91736, #121190, #11227 ) ;
#33414=ORIENTED_EDGE ( 'NONE', *, *, #104583, .T. ) ;
#33415=CARTESIAN_POINT ( 'NONE',  ( -6.850000000000013856, 12.50000000000000000, 6.148780366869520897 ) ) ;
#33417=ORIENTED_EDGE ( 'NONE', *, *, #66418, .F. ) ;
#33418=CARTESIAN_POINT ( 'NONE',  ( 3.749999999999944045, 12.50000000000000000, -7.253104124594891289 ) ) ;
#33419=DIRECTION ( 'NONE',  ( -4.274815082592931898E-19, -0.9999939076577903929, -0.003490651415223739937 ) ) ;
#33420=CARTESIAN_POINT ( 'NONE',  ( -6.650000000000019007, 2.500000000000000000, -1.472243186433550122 ) ) ;
#33421=EDGE_CURVE ( 'NONE', #115634, #77218, #108981, .T. ) ;
#33423=CARTESIAN_POINT ( 'NONE',  ( -10.40000000000000213, 2.500000000000000000, 0.09999999999999772959 ) ) ;
#33424=DIRECTION ( 'NONE',  ( -4.274815082592931898E-19, -0.9999939076577903929, -0.003490651415223739937 ) ) ;
#33425=CARTESIAN_POINT ( 'NONE',  ( -8.750000000000008882, 12.50000000000000000, 1.472243186433545459 ) ) ;
#33426=ORIENTED_EDGE ( 'NONE', *, *, #11738, .T. ) ;
#33427=DIRECTION ( 'NONE',  ( -0.000000000000000000, -1.000000000000000000, -0.000000000000000000 ) ) ;
#33428=DIRECTION ( 'NONE',  ( 0.000000000000000000, 0.000000000000000000, 1.000000000000000000 ) ) ;
#33429=VERTEX_POINT ( 'NONE', #117136 ) ;
#33430=AXIS2_PLACEMENT_3D ( 'NONE', #54520, #23140, #74178 ) ;
#33431=AXIS2_PLACEMENT_3D ( 'NONE', #28599, #116954, #38434 ) ;
#33432=ORIENTED_EDGE ( 'NONE', *, *, #89424, .F. ) ;
#33433=ORIENTED_EDGE ( 'NONE', *, *, #66831, .T. ) ;
#33434=EDGE_CURVE ( 'NONE', #75499, #129204, #113190, .T. ) ;
#33435=EDGE_CURVE ( 'NONE', #117286, #72026, #88131, .T. ) ;
#33436=VERTEX_POINT ( 'NONE', #75298 ) ;
#33437=DIRECTION ( 'NONE',  ( 0.000000000000000000, 1.000000000000000000, 0.000000000000000000 ) ) ;
#33438=DIRECTION ( 'NONE',  ( 0.000000000000000000, 0.000000000000000000, -1.000000000000000000 ) ) ;
#33439=CIRCLE ( 'NONE', #6209, 0.1000000000000000472 ) ;
#33440=AXIS2_PLACEMENT_3D ( 'NONE', #119192, #50445, #9882 ) ;
#33441=DIRECTION ( 'NONE',  ( -0.000000000000000000, -1.000000000000000000, -0.000000000000000000 ) ) ;
#33442=DIRECTION ( 'NONE',  ( -0.000000000000000000, -1.000000000000000000, -0.000000000000000000 ) ) ;
#33443=DIRECTION ( 'NONE',  ( 0.000000000000000000, 0.000000000000000000, -1.000000000000000000 ) ) ;
#33444=ORIENTED_EDGE ( 'NONE', *, *, #22473, .F. ) ;
#33445=LINE ( 'NONE', #114550, #99613 ) ;
#33447=CARTESIAN_POINT ( 'NONE',  ( -2.300000000000033573, 2.500000000000000000, 0.3464101615137735735 ) ) ;
#33448=CARTESIAN_POINT ( 'NONE',  ( -8.100000000000010303, 2.500000000000000000, 4.776537180435972196 ) ) ;
#33450=CIRCLE ( 'NONE', #85657, 0.09999999999999982514 ) ;
#33451=EDGE_LOOP ( 'NONE', ( #23721, #35786, #107268, #50136 ) ) ;
#33452=AXIS2_PLACEMENT_3D ( 'NONE', #53112, #55678, #64206 ) ;
#33453=VERTEX_POINT ( 'NONE', #70007 ) ;
#33454=ORIENTED_EDGE ( 'NONE', *, *, #92132, .F. ) ;
#33455=FACE_OUTER_BOUND ( 'NONE', #114301, .T. ) ;
#33456=VECTOR ( 'NONE', #58332, 1000.000000000000000 ) ;
#33457=AXIS2_PLACEMENT_3D ( 'NONE', #45680, #86217, #46972 ) ;
#33458=CARTESIAN_POINT ( 'NONE',  ( 7.099999999999927702, 2.500000000000000000, 5.122947341949749323 ) ) ;
#33459=DIRECTION ( 'NONE',  ( 0.000000000000000000, 1.000000000000000000, 0.000000000000000000 ) ) ;
#33460=CONICAL_SURFACE ( 'NONE', #119218, 0.1000000000000002554, 0.003490658503988666988 ) ;
#33461=ORIENTED_EDGE ( 'NONE', *, *, #7085, .T. ) ;
#33462=LINE ( 'NONE', #22357, #101745 ) ;
#33463=LINE ( 'NONE', #104122, #20407 ) ;
#33464=FACE_OUTER_BOUND ( 'NONE', #25258, .T. ) ;
#33465=DIRECTION ( 'NONE',  ( -4.274815082592931898E-19, -0.9999939076577903929, -0.003490651415223739937 ) ) ;
#33466=ADVANCED_FACE ( 'NONE', ( #79190 ), #119730, .T. ) ;
#33467=CARTESIAN_POINT ( 'NONE',  ( 11.24999999999994316, 12.50000000000000000, -6.495190528383302464 ) ) ;
#33468=VERTEX_POINT ( 'NONE', #28794 ) ;
#33469=VERTEX_POINT ( 'NONE', #68701 ) ;
#33470=ADVANCED_FACE ( 'NONE', ( #99472 ), #83947, .T. ) ;
#33471=CARTESIAN_POINT ( 'NONE',  ( 0.5999999999999547917, 2.500000000000000000, 4.083716857408420609 ) ) ;
#33472=CARTESIAN_POINT ( 'NONE',  ( -13.74999999999998934, 12.50000000000000000, 2.857883832488652853 ) ) ;
#33473=ADVANCED_FACE ( 'NONE', ( #18308 ), #119452, .T. ) ;
#33474=DIRECTION ( 'NONE',  ( -0.000000000000000000, 1.000000000000000000, -0.000000000000000000 ) ) ;
#33475=PLANE ( 'NONE',  #63222 ) ;
#33476=DIRECTION ( 'NONE',  ( 0.000000000000000000, 0.000000000000000000, -1.000000000000000000 ) ) ;
#33477=ORIENTED_EDGE ( 'NONE', *, *, #82971, .F. ) ;
#33478=EDGE_CURVE ( 'NONE', #37568, #76503, #123646, .T. ) ;
#33479=EDGE_CURVE ( 'NONE', #48393, #29366, #48452, .T. ) ;
#33480=VERTEX_POINT ( 'NONE', #10428 ) ;
#33481=CARTESIAN_POINT ( 'NONE',  ( -4.600000000000024514, 2.500000000000000000, 5.022947341949748790 ) ) ;
#33483=DIRECTION ( 'NONE',  ( 0.000000000000000000, 1.000000000000000000, 0.000000000000000000 ) ) ;
#33484=EDGE_CURVE ( 'NONE', #126271, #98359, #98798, .T. ) ;
#33485=DIRECTION ( 'NONE',  ( 0.000000000000000000, 1.000000000000000000, 0.000000000000000000 ) ) ;
#33486=LINE ( 'NONE', #15586, #64375 ) ;
#33487=CARTESIAN_POINT ( 'NONE',  ( -5.850000000000022737, 2.500000000000000000, -2.065063509461102065 ) ) ;
#33488=ORIENTED_EDGE ( 'NONE', *, *, #55189, .F. ) ;
#33489=PLANE ( 'NONE',  #2966 ) ;
#33490=CIRCLE ( 'NONE', #85780, 0.06509327318403741736 ) ;
#33491=CIRCLE ( 'NONE', #106628, 0.09999999999999982514 ) ;
#33492=EDGE_CURVE ( 'NONE', #116919, #22551, #29437, .T. ) ;
#33493=DIRECTION ( 'NONE',  ( 0.000000000000000000, 0.000000000000000000, 1.000000000000000000 ) ) ;
#33494=EDGE_LOOP ( 'NONE', ( #68866, #32905 ) ) ;
#33495=DIRECTION ( 'NONE',  ( 0.000000000000000000, 0.000000000000000000, 1.000000000000000000 ) ) ;
#33496=ORIENTED_EDGE ( 'NONE', *, *, #7799, .F. ) ;
#33497=EDGE_CURVE ( 'NONE', #19146, #125479, #52565, .T. ) ;
#33498=FACE_OUTER_BOUND ( 'NONE', #106778, .T. ) ;
#33499=CIRCLE ( 'NONE', #8337, 0.06509327318403745899 ) ;
#33500=ORIENTED_EDGE ( 'NONE', *, *, #114910, .T. ) ;
#33501=CARTESIAN_POINT ( 'NONE',  ( 5.599999999999934808, 12.50000000000000000, -3.983716857408426293 ) ) ;
#33502=FACE_OUTER_BOUND ( 'NONE', #38657, .T. ) ;
#33503=ORIENTED_EDGE ( 'NONE', *, *, #127988, .T. ) ;
#33504=ORIENTED_EDGE ( 'NONE', *, *, #27658, .F. ) ;
#33506=FACE_OUTER_BOUND ( 'NONE', #31939, .T. ) ;
#33509=DIRECTION ( 'NONE',  ( 0.000000000000000000, 0.000000000000000000, 1.000000000000000000 ) ) ;
#33510=DIRECTION ( 'NONE',  ( -0.000000000000000000, 1.000000000000000000, -0.000000000000000000 ) ) ;
#33511=DIRECTION ( 'NONE',  ( 0.000000000000000000, -0.000000000000000000, 1.000000000000000000 ) ) ;
#33512=LINE ( 'NONE', #80676, #127906 ) ;
#33513=CIRCLE ( 'NONE', #12648, 0.06509327318403745899 ) ;
#33514=AXIS2_PLACEMENT_3D ( 'NONE', #63792, #25136, #65048 ) ;
#33515=ORIENTED_EDGE ( 'NONE', *, *, #115871, .T. ) ;
#33516=EDGE_LOOP ( 'NONE', ( #38244, #110882, #76451, #23820 ) ) ;
#33517=DIRECTION ( 'NONE',  ( 0.000000000000000000, -0.9999939076577903929, 0.003490651415223739937 ) ) ;
#33518=ORIENTED_EDGE ( 'NONE', *, *, #71669, .T. ) ;
#33519=DIRECTION ( 'NONE',  ( 0.000000000000000000, 0.000000000000000000, 1.000000000000000000 ) ) ;
#33520=CARTESIAN_POINT ( 'NONE',  ( -1.850000000000033840, 12.50000000000000000, 1.883746621131358934 ) ) ;
#33521=DIRECTION ( 'NONE',  ( -4.274815082592931898E-19, -0.9999939076577903929, -0.003490651415223739937 ) ) ;
#33522=ORIENTED_EDGE ( 'NONE', *, *, #16974, .F. ) ;
#33523=VERTEX_POINT ( 'NONE', #87691 ) ;
#33524=FACE_BOUND ( 'NONE', #115516, .T. ) ;
#33525=ORIENTED_EDGE ( 'NONE', *, *, #73303, .T. ) ;
#33526=DIRECTION ( 'NONE',  ( 0.000000000000000000, 0.000000000000000000, 1.000000000000000000 ) ) ;
#33528=AXIS2_PLACEMENT_3D ( 'NONE', #24120, #64041, #103971 ) ;
#33529=FACE_OUTER_BOUND ( 'NONE', #125506, .T. ) ;
#33530=DIRECTION ( 'NONE',  ( -0.000000000000000000, 1.000000000000000000, -0.000000000000000000 ) ) ;
#33531=EDGE_CURVE ( 'NONE', #109159, #69422, #125701, .T. ) ;
#33532=CARTESIAN_POINT ( 'NONE',  ( -8.950000000000008171, 2.500000000000000000, -2.511473670974877948 ) ) ;
#33533=CARTESIAN_POINT ( 'NONE',  ( 2.499999999999947153, 12.50000000000000000, 0.6928203230275494784 ) ) ;
#33534=DIRECTION ( 'NONE',  ( -0.000000000000000000, 1.000000000000000000, -0.000000000000000000 ) ) ;
#33536=CARTESIAN_POINT ( 'NONE',  ( 4.149999999999938183, 2.500000000000000000, 5.702370205355745014 ) ) ;
#33537=DIRECTION ( 'NONE',  ( 0.000000000000000000, 0.000000000000000000, -1.000000000000000000 ) ) ;
#33538=AXIS2_PLACEMENT_3D ( 'NONE', #70509, #51536, #43025 ) ;
#33539=DIRECTION ( 'NONE',  ( -0.000000000000000000, 1.000000000000000000, -0.000000000000000000 ) ) ;
#33541=CONICAL_SURFACE ( 'NONE', #123399, 0.09999999999999982514, 0.003490658503988666988 ) ;
#33542=ORIENTED_EDGE ( 'NONE', *, *, #99780, .T. ) ;
#33543=ORIENTED_EDGE ( 'NONE', *, *, #7721, .T. ) ;
#33544=VECTOR ( 'NONE', #26065, 1000.000000000000000 ) ;
#33545=ORIENTED_EDGE ( 'NONE', *, *, #96812, .T. ) ;
#33546=DIRECTION ( 'NONE',  ( 0.000000000000000000, 1.000000000000000000, 0.000000000000000000 ) ) ;
#33547=EDGE_LOOP ( 'NONE', ( #56693, #85440, #112923, #114681 ) ) ;
#33548=LINE ( 'NONE', #45776, #67439 ) ;
#33549=ORIENTED_EDGE ( 'NONE', *, *, #104056, .F. ) ;
#33550=VERTEX_POINT ( 'NONE', #97515 ) ;
#33551=ORIENTED_EDGE ( 'NONE', *, *, #26493, .T. ) ;
#33553=VECTOR ( 'NONE', #55670, 1000.000000000000000 ) ;
#33554=FACE_OUTER_BOUND ( 'NONE', #53552, .T. ) ;
#33555=DIRECTION ( 'NONE',  ( 0.000000000000000000, 0.000000000000000000, -1.000000000000000000 ) ) ;
#33556=AXIS2_PLACEMENT_3D ( 'NONE', #630, #51051, #40602 ) ;
#33557=LINE ( 'NONE', #53822, #74859 ) ;
#33558=CARTESIAN_POINT ( 'NONE',  ( 9.149999999999920419, 2.500000000000000000, 2.857883832488649301 ) ) ;
#33559=ORIENTED_EDGE ( 'NONE', *, *, #68202, .T. ) ;
#33560=DIRECTION ( 'NONE',  ( -0.000000000000000000, 1.000000000000000000, -0.000000000000000000 ) ) ;
#33561=ORIENTED_EDGE ( 'NONE', *, *, #54930, .F. ) ;
#33563=ORIENTED_EDGE ( 'NONE', *, *, #68480, .T. ) ;
#33564=DIRECTION ( 'NONE',  ( 0.000000000000000000, 1.000000000000000000, 0.000000000000000000 ) ) ;
#33565=ORIENTED_EDGE ( 'NONE', *, *, #19870, .T. ) ;
#33566=EDGE_LOOP ( 'NONE', ( #68091, #70742 ) ) ;
#33567=VERTEX_POINT ( 'NONE', #110563 ) ;
#33568=CARTESIAN_POINT ( 'NONE',  ( -1.450000000000036371, 2.500000000000000000, 6.941600689897073018 ) ) ;
#33569=ADVANCED_FACE ( 'NONE', ( #58257 ), #96463, .T. ) ;
#33570=DIRECTION ( 'NONE',  ( 0.000000000000000000, -0.9999939076577903929, 0.003490651415223739937 ) ) ;
#33571=DIRECTION ( 'NONE',  ( 0.000000000000000000, -0.000000000000000000, 1.000000000000000000 ) ) ;
#33572=CARTESIAN_POINT ( 'NONE',  ( -5.400000000000023448, 2.500000000000000000, -5.022947341949754119 ) ) ;
#33573=DIRECTION ( 'NONE',  ( 0.000000000000000000, 0.000000000000000000, -1.000000000000000000 ) ) ;
#33574=CIRCLE ( 'NONE', #94109, 0.06509327318403745899 ) ;
#33575=DIRECTION ( 'NONE',  ( 0.000000000000000000, 1.000000000000000000, 0.000000000000000000 ) ) ;
#33576=CONICAL_SURFACE ( 'NONE', #48143, 0.09999999999999982514, 0.003490658503988666988 ) ;
#33577=DIRECTION ( 'NONE',  ( 0.000000000000000000, 1.000000000000000000, 0.000000000000000000 ) ) ;
#33578=ADVANCED_FACE ( 'NONE', ( #20254 ), #75537, .T. ) ;
#33579=EDGE_LOOP ( 'NONE', ( #39934, #24717 ) ) ;
#33580=CARTESIAN_POINT ( 'NONE',  ( 11.44999999999991047, 2.500000000000000000, 6.048780366869520364 ) ) ;
#33581=AXIS2_PLACEMENT_3D ( 'NONE', #11378, #12018, #259 ) ;
#33582=ORIENTED_EDGE ( 'NONE', *, *, #8577, .T. ) ;
#33583=CARTESIAN_POINT ( 'NONE',  ( -1.850000000000033840, 12.50000000000000000, 6.148780366869520897 ) ) ;
#33584=VERTEX_POINT ( 'NONE', #68056 ) ;
#33585=EDGE_CURVE ( 'NONE', #32548, #63751, #129590, .T. ) ;
#33586=EDGE_CURVE ( 'NONE', #100700, #37856, #104871, .T. ) ;
#33587=ORIENTED_EDGE ( 'NONE', *, *, #41637, .F. ) ;
#33588=DIRECTION ( 'NONE',  ( 0.000000000000000000, 0.000000000000000000, 1.000000000000000000 ) ) ;
#33589=DIRECTION ( 'NONE',  ( 0.000000000000000000, 0.000000000000000000, -1.000000000000000000 ) ) ;
#33590=ADVANCED_FACE ( 'NONE', ( #77868 ), #94412, .T. ) ;
#33591=DIRECTION ( 'NONE',  ( -0.000000000000000000, 1.000000000000000000, -0.000000000000000000 ) ) ;
#33592=EDGE_LOOP ( 'NONE', ( #103117, #91828 ) ) ;
#33593=EDGE_LOOP ( 'NONE', ( #74915, #51920 ) ) ;
#33594=CARTESIAN_POINT ( 'NONE',  ( -12.89999999999999147, 12.50000000000000000, 1.843143693225357538E-15 ) ) ;
#33595=CARTESIAN_POINT ( 'NONE',  ( 2.500000000000002220, -0.5000000000000000000, -9.999999999999998224 ) ) ;
#33596=ADVANCED_FACE ( 'NONE', ( #128289 ), #14965, .T. ) ;
#33597=DIRECTION ( 'NONE',  ( 0.000000000000000000, 1.000000000000000000, 0.000000000000000000 ) ) ;
#33598=DIRECTION ( 'NONE',  ( -0.000000000000000000, -1.000000000000000000, -0.000000000000000000 ) ) ;
#33599=DIRECTION ( 'NONE',  ( 0.000000000000000000, 1.000000000000000000, 0.000000000000000000 ) ) ;
#33600=ORIENTED_EDGE ( 'NONE', *, *, #44319, .T. ) ;
#33601=ORIENTED_EDGE ( 'NONE', *, *, #103920, .T. ) ;
#33602=DIRECTION ( 'NONE',  ( 0.000000000000000000, 1.000000000000000000, 0.000000000000000000 ) ) ;
#33603=CIRCLE ( 'NONE', #106735, 0.1000000000000002554 ) ;
#33604=FACE_OUTER_BOUND ( 'NONE', #4357, .T. ) ;
#33605=VECTOR ( 'NONE', #41788, 1000.000000000000000 ) ;
#33607=DIRECTION ( 'NONE',  ( -0.000000000000000000, 1.000000000000000000, -0.000000000000000000 ) ) ;
#33608=FACE_OUTER_BOUND ( 'NONE', #12244, .T. ) ;
#33609=DIRECTION ( 'NONE',  ( 0.000000000000000000, 1.000000000000000000, 0.000000000000000000 ) ) ;
#33610=DIRECTION ( 'NONE',  ( -0.000000000000000000, -1.000000000000000000, -0.000000000000000000 ) ) ;
#33611=ORIENTED_EDGE ( 'NONE', *, *, #20141, .F. ) ;
#33612=AXIS2_PLACEMENT_3D ( 'NONE', #8968, #48924, #88828 ) ;
#33613=CARTESIAN_POINT ( 'NONE',  ( 6.449999999999931788, 12.50000000000000000, -2.576566944158915184 ) ) ;
#33614=ADVANCED_FACE ( 'NONE', ( #71947 ), #111193, .T. ) ;
#33615=CARTESIAN_POINT ( 'NONE',  ( -4.600000000000025402, 2.500000000000000000, 4.230127018922196669 ) ) ;
#33616=CARTESIAN_POINT ( 'NONE',  ( 10.44999999999991047, 2.500000000000000000, 2.165063509461097713 ) ) ;
#33617=ORIENTED_EDGE ( 'NONE', *, *, #60539, .T. ) ;
#33618=EDGE_CURVE ( 'NONE', #118696, #62991, #92261, .T. ) ;
#33619=DIRECTION ( 'NONE',  ( 0.000000000000000000, 1.000000000000000000, 0.000000000000000000 ) ) ;
#33620=CONICAL_SURFACE ( 'NONE', #16854, 0.1000000000000002554, 0.003490658503988666988 ) ;
#33621=ORIENTED_EDGE ( 'NONE', *, *, #39935, .F. ) ;
#33622=PRODUCT ( 'Brush Head Assembly', 'Brush Head Assembly', '', ( #26784 ) ) ;
#33623=DIRECTION ( 'NONE',  ( 0.000000000000000000, 1.000000000000000000, 0.000000000000000000 ) ) ;
#33624=EDGE_CURVE ( 'NONE', #40211, #59797, #35847, .T. ) ;
#33625=ORIENTED_EDGE ( 'NONE', *, *, #45133, .F. ) ;
#33626=DIRECTION ( 'NONE',  ( 0.000000000000000000, -0.000000000000000000, 1.000000000000000000 ) ) ;
#33627=DIRECTION ( 'NONE',  ( 0.000000000000000000, 0.000000000000000000, 1.000000000000000000 ) ) ;
#33628=EDGE_CURVE ( 'NONE', #129270, #77431, #17014, .T. ) ;
#33630=AXIS2_PLACEMENT_3D ( 'NONE', #37815, #69859, #18811 ) ;
#33631=ADVANCED_FACE ( 'NONE', ( #83055 ), #12826, .T. ) ;
#33633=LINE ( 'NONE', #113471, #76028 ) ;
#33634=ADVANCED_FACE ( 'NONE', ( #111866 ), #85994, .T. ) ;
#33635=DIRECTION ( 'NONE',  ( -0.000000000000000000, 1.000000000000000000, -0.000000000000000000 ) ) ;
#33636=CIRCLE ( 'NONE', #121355, 0.06509327318403745899 ) ;
#33637=VERTEX_POINT ( 'NONE', #32028 ) ;
#33638=ADVANCED_FACE ( 'NONE', ( #63404 ), #113797, .T. ) ;
#33639=ADVANCED_FACE ( 'NONE', ( #60828 ), #21258, .T. ) ;
#33640=EDGE_LOOP ( 'NONE', ( #975, #46832 ) ) ;
#33641=VERTEX_POINT ( 'NONE', #72587 ) ;
#33642=DIRECTION ( 'NONE',  ( -0.000000000000000000, -1.000000000000000000, -0.000000000000000000 ) ) ;
#33643=FACE_OUTER_BOUND ( 'NONE', #33579, .T. ) ;
#33644=DIRECTION ( 'NONE',  ( 0.000000000000000000, 1.000000000000000000, 0.000000000000000000 ) ) ;
#33645=ORIENTED_EDGE ( 'NONE', *, *, #80297, .T. ) ;
#33646=FACE_OUTER_BOUND ( 'NONE', #2266, .T. ) ;
#33648=ORIENTED_EDGE ( 'NONE', *, *, #47928, .F. ) ;
#33649=DIRECTION ( 'NONE',  ( 0.000000000000000000, 0.000000000000000000, 1.000000000000000000 ) ) ;
#33650=CARTESIAN_POINT ( 'NONE',  ( -1.250000000000035749, 2.500000000000000000, -2.957883832488653830 ) ) ;
#33651=VECTOR ( 'NONE', #94246, 1000.000000000000000 ) ;
#33652=DIRECTION ( 'NONE',  ( -0.000000000000000000, -1.000000000000000000, -0.000000000000000000 ) ) ;
#33654=DIRECTION ( 'NONE',  ( 0.000000000000000000, -0.000000000000000000, 1.000000000000000000 ) ) ;
#33655=CIRCLE ( 'NONE', #123523, 0.1000000000000002554 ) ;
#33656=AXIS2_PLACEMENT_3D ( 'NONE', #39699, #79594, #119504 ) ;
#33657=DIRECTION ( 'NONE',  ( 0.000000000000000000, 0.000000000000000000, 1.000000000000000000 ) ) ;
#33658=DIRECTION ( 'NONE',  ( 0.000000000000000000, 0.000000000000000000, -1.000000000000000000 ) ) ;
#33659=AXIS2_PLACEMENT_3D ( 'NONE', #38786, #100885, #91075 ) ;
#33660=ORIENTED_EDGE ( 'NONE', *, *, #10409, .F. ) ;
#33661=ORIENTED_EDGE ( 'NONE', *, *, #23881, .T. ) ;
#33662=ORIENTED_EDGE ( 'NONE', *, *, #41680, .F. ) ;
#33664=CARTESIAN_POINT ( 'NONE',  ( 3.949999999999941558, 2.500000000000000000, -1.718653347947326049 ) ) ;
#33665=CARTESIAN_POINT ( 'NONE',  ( 0.6499999999999561684, 12.50000000000000000, 1.818653347947321475 ) ) ;
#33666=AXIS2_PLACEMENT_3D ( 'NONE', #53354, #21296, #12750 ) ;
#33667=DIRECTION ( 'NONE',  ( -4.274815082592931898E-19, -0.9999939076577903929, -0.003490651415223739937 ) ) ;
#33669=FACE_BOUND ( 'NONE', #84031, .T. ) ;
#33670=DIRECTION ( 'NONE',  ( -0.000000000000000000, -1.000000000000000000, -0.000000000000000000 ) ) ;
#33671=CARTESIAN_POINT ( 'NONE',  ( 3.549999999999942979, 12.50000000000000000, 1.883746621131358934 ) ) ;
#33672=CARTESIAN_POINT ( 'NONE',  ( 10.59999999999991260, 12.50000000000000000, -0.3464101615137783474 ) ) ;
#33673=ADVANCED_FACE ( 'NONE', ( #62768 ), #50503, .T. ) ;
#33674=CARTESIAN_POINT ( 'NONE',  ( 8.349999999999923261, 2.500000000000000000, -5.802370205355749988 ) ) ;
#33675=PLANE ( 'NONE',  #32631 ) ;
#33676=DIRECTION ( 'NONE',  ( 0.000000000000000000, 0.000000000000000000, 1.000000000000000000 ) ) ;
#33677=FACE_OUTER_BOUND ( 'NONE', #41190, .T. ) ;
#33678=CARTESIAN_POINT ( 'NONE',  ( -1.850000000000033840, 12.50000000000000000, 6.148780366869520897 ) ) ;
#33679=CARTESIAN_POINT ( 'NONE',  ( 14.34999999999989662, 12.50000000000000000, 2.446380397790835826 ) ) ;
#33680=FACE_OUTER_BOUND ( 'NONE', #44230, .T. ) ;
#33681=EDGE_LOOP ( 'NONE', ( #122256, #103792, #30286, #24965 ) ) ;
#33682=EDGE_CURVE ( 'NONE', #102865, #85037, #106930, .T. ) ;
#33683=AXIS2_PLACEMENT_3D ( 'NONE', #37246, #88231, #106604 ) ;
#33684=ORIENTED_EDGE ( 'NONE', *, *, #68210, .F. ) ;
#33685=ORIENTED_EDGE ( 'NONE', *, *, #68890, .F. ) ;
#33686=ORIENTED_EDGE ( 'NONE', *, *, #28330, .F. ) ;
#33687=ORIENTED_EDGE ( 'NONE', *, *, #37719, .T. ) ;
#33688=ORIENTED_EDGE ( 'NONE', *, *, #31412, .T. ) ;
#33689=DIRECTION ( 'NONE',  ( 0.000000000000000000, 0.000000000000000000, -1.000000000000000000 ) ) ;
#33690=EDGE_LOOP ( 'NONE', ( #23147, #53986 ) ) ;
#33691=VERTEX_POINT ( 'NONE', #51664 ) ;
#33692=AXIS2_PLACEMENT_3D ( 'NONE', #21516, #90231, #80442 ) ;
#33693=CARTESIAN_POINT ( 'NONE',  ( 15.40585131749378967, -2.500000000000000444, 5.817868756321115775 ) ) ;
#33694=DIRECTION ( 'NONE',  ( -0.000000000000000000, 1.000000000000000000, -0.000000000000000000 ) ) ;
#33695=FACE_OUTER_BOUND ( 'NONE', #10719, .T. ) ;
#33696=VERTEX_POINT ( 'NONE', #102671 ) ;
#33697=CARTESIAN_POINT ( 'NONE',  ( -6.450000000000017941, 2.500000000000000000, -6.841600689897077814 ) ) ;
#33698=AXIS2_PLACEMENT_3D ( 'NONE', #20530, #30362, #71548 ) ;
#33700=EDGE_LOOP ( 'NONE', ( #119316, #119799 ) ) ;
#33701=DIRECTION ( 'NONE',  ( 0.000000000000000000, 1.000000000000000000, 0.000000000000000000 ) ) ;
#33702=LINE ( 'NONE', #73615, #83917 ) ;
#33703=ORIENTED_EDGE ( 'NONE', *, *, #118878, .F. ) ;
#33704=ORIENTED_EDGE ( 'NONE', *, *, #41419, .T. ) ;
#33705=CIRCLE ( 'NONE', #60891, 0.06509327318403745899 ) ;
#33707=VECTOR ( 'NONE', #37018, 1000.000000000000000 ) ;
#33708=PLANE ( 'NONE',  #101805 ) ;
#33709=CARTESIAN_POINT ( 'NONE',  ( 7.949999999999922018, 2.500000000000000000, 6.495190528383297135 ) ) ;
#33711=DIRECTION ( 'NONE',  ( 0.000000000000000000, 0.000000000000000000, 1.000000000000000000 ) ) ;
#33712=CIRCLE ( 'NONE', #106853, 0.06509327318403743123 ) ;
#33713=ORIENTED_EDGE ( 'NONE', *, *, #99772, .F. ) ;
#33714=FACE_OUTER_BOUND ( 'NONE', #88250, .T. ) ;
#33715=ADVANCED_FACE ( 'NONE', ( #12988 ), #52941, .T. ) ;
#33716=ORIENTED_EDGE ( 'NONE', *, *, #103507, .F. ) ;
#33717=CARTESIAN_POINT ( 'NONE',  ( 17.50000000000000000, 2.499999999999999556, 1.666666666666669849 ) ) ;
#33718=ORIENTED_EDGE ( 'NONE', *, *, #28255, .T. ) ;
#33719=DIRECTION ( 'NONE',  ( -0.000000000000000000, -1.000000000000000000, -0.000000000000000000 ) ) ;
#33720=CIRCLE ( 'NONE', #83796, 0.1000000000000002554 ) ;
#33721=AXIS2_PLACEMENT_3D ( 'NONE', #3138, #114363, #13578 ) ;
#33722=DIRECTION ( 'NONE',  ( 0.000000000000000000, 0.000000000000000000, 1.000000000000000000 ) ) ;
#33724=EDGE_CURVE ( 'NONE', #11464, #75789, #19187, .T. ) ;
#33726=EDGE_CURVE ( 'NONE', #24379, #99999, #73861, .T. ) ;
#33727=EDGE_LOOP ( 'NONE', ( #91395, #123213, #57864, #95921 ) ) ;
#33728=EDGE_CURVE ( 'NONE', #74675, #92671, #67284, .T. ) ;
#33729=CARTESIAN_POINT ( 'NONE',  ( -1.250000000000001110, 12.50000000000000000, -6.560283801567339701 ) ) ;
#33730=VERTEX_POINT ( 'NONE', #91571 ) ;
#33731=ADVANCED_FACE ( 'NONE', ( #81740 ), #28406, .T. ) ;
#33732=ORIENTED_EDGE ( 'NONE', *, *, #53835, .T. ) ;
#33733=EDGE_LOOP ( 'NONE', ( #64446, #2153 ) ) ;
#33734=DIRECTION ( 'NONE',  ( 0.000000000000000000, -0.000000000000000000, 1.000000000000000000 ) ) ;
#33735=DIRECTION ( 'NONE',  ( -0.000000000000000000, -1.000000000000000000, -0.000000000000000000 ) ) ;
#33736=EDGE_CURVE ( 'NONE', #83877, #14873, #124260, .T. ) ;
#33738=DIRECTION ( 'NONE',  ( 0.000000000000000000, -0.000000000000000000, 1.000000000000000000 ) ) ;
#33739=DIRECTION ( 'NONE',  ( 1.000000000000000000, 0.000000000000000000, 0.000000000000000000 ) ) ;
#33740=DIRECTION ( 'NONE',  ( 0.000000000000000000, 1.000000000000000000, 0.000000000000000000 ) ) ;
#33741=AXIS2_PLACEMENT_3D ( 'NONE', #75894, #67330, #16936 ) ;
#33742=VECTOR ( 'NONE', #68825, 1000.000000000000000 ) ;
#33743=AXIS2_PLACEMENT_3D ( 'NONE', #47410, #48054, #88613 ) ;
#33744=ORIENTED_EDGE ( 'NONE', *, *, #25692, .F. ) ;
#33745=CARTESIAN_POINT ( 'NONE',  ( -1.650000000000034328, 2.500000000000000000, -2.265063509461101798 ) ) ;
#33746=VECTOR ( 'NONE', #13789, 1000.000000000000000 ) ;
#33747=AXIS2_PLACEMENT_3D ( 'NONE', #66519, #75691, #25294 ) ;
#33748=VERTEX_POINT ( 'NONE', #103976 ) ;
#33749=DIRECTION ( 'NONE',  ( 0.000000000000000000, -0.000000000000000000, 1.000000000000000000 ) ) ;
#33750=CONICAL_SURFACE ( 'NONE', #115190, 0.1000000000000002554, 0.003490658503988666988 ) ;
#33751=LINE ( 'NONE', #4266, #74465 ) ;
#33752=FACE_OUTER_BOUND ( 'NONE', #34322, .T. ) ;
#33753=DIRECTION ( 'NONE',  ( 0.000000000000000000, 0.000000000000000000, -1.000000000000000000 ) ) ;
#33754=ORIENTED_EDGE ( 'NONE', *, *, #99567, .T. ) ;
#33755=CARTESIAN_POINT ( 'NONE',  ( 2.299999999999948752, 2.500000000000000000, 0.2464101615137735679 ) ) ;
#33756=DIRECTION ( 'NONE',  ( -0.000000000000000000, -1.000000000000000000, -0.000000000000000000 ) ) ;
#33757=ORIENTED_EDGE ( 'NONE', *, *, #36573, .T. ) ;
#33758=ORIENTED_EDGE ( 'NONE', *, *, #53586, .T. ) ;
#33759=DIRECTION ( 'NONE',  ( 0.000000000000000000, 0.000000000000000000, 1.000000000000000000 ) ) ;
#33760=EDGE_LOOP ( 'NONE', ( #30905, #80490, #110088, #64501 ) ) ;
#33761=ORIENTED_EDGE ( 'NONE', *, *, #51797, .F. ) ;
#33762=DIRECTION ( 'NONE',  ( -0.000000000000000000, -1.000000000000000000, -0.000000000000000000 ) ) ;
#33763=ADVANCED_FACE ( 'NONE', ( #34612 ), #95443, .T. ) ;
#33764=EDGE_CURVE ( 'NONE', #58977, #77164, #104605, .T. ) ;
#33765=ORIENTED_EDGE ( 'NONE', *, *, #124792, .T. ) ;
#33766=CARTESIAN_POINT ( 'NONE',  ( 15.86953761860682910, 2.463355995079617333, -3.896699429476665699 ) ) ;
#33767=CARTESIAN_POINT ( 'NONE',  ( -4.600000000000024514, 12.50000000000000000, 0.6928203230275494784 ) ) ;
#33768=EDGE_CURVE ( 'NONE', #108142, #62304, #65976, .T. ) ;
#33769=LINE ( 'NONE', #4283, #8154 ) ;
#33770=CIRCLE ( 'NONE', #83936, 0.1000000000000000056 ) ;
#33771=ORIENTED_EDGE ( 'NONE', *, *, #123260, .F. ) ;
#33772=ADVANCED_FACE ( 'NONE', ( #96711 ), #44336, .T. ) ;
#33773=DIRECTION ( 'NONE',  ( 0.000000000000000000, 0.000000000000000000, -1.000000000000000000 ) ) ;
#33775=ORIENTED_EDGE ( 'NONE', *, *, #16275, .F. ) ;
#33776=ADVANCED_FACE ( 'NONE', ( #124901 ), #98604, .T. ) ;
#33777=DIRECTION ( 'NONE',  ( -4.274815082592931898E-19, -0.9999939076577903929, -0.003490651415223739937 ) ) ;
#33778=EDGE_CURVE ( 'NONE', #29034, #67278, #31825, .T. ) ;
#33779=CARTESIAN_POINT ( 'NONE',  ( 10.59999999999990905, 2.500000000000000000, -4.676537180435978769 ) ) ;
#33780=EDGE_LOOP ( 'NONE', ( #56773, #124817, #93411, #40649 ) ) ;
#33782=ADVANCED_FACE ( 'NONE', ( #8334 ), #38470, .T. ) ;
#33783=EDGE_CURVE ( 'NONE', #50249, #124819, #21352, .T. ) ;
#33784=AXIS2_PLACEMENT_3D ( 'NONE', #27293, #59374, #69813 ) ;
#33785=ORIENTED_EDGE ( 'NONE', *, *, #14444, .F. ) ;
#33786=ORIENTED_EDGE ( 'NONE', *, *, #112362, .T. ) ;
#33787=EDGE_LOOP ( 'NONE', ( #38540, #7121 ) ) ;
#33788=CARTESIAN_POINT ( 'NONE',  ( 4.149999999999941735, 2.500000000000000000, -1.472243186433550122 ) ) ;
#33789=CARTESIAN_POINT ( 'NONE',  ( 3.709550432145489740, 2.499999999999999556, 9.999999999907080550 ) ) ;
#33790=DIRECTION ( 'NONE',  ( -0.000000000000000000, 1.000000000000000000, -0.000000000000000000 ) ) ;
#33791=FACE_BOUND ( 'NONE', #4132, .T. ) ;
#33792=EDGE_LOOP ( 'NONE', ( #99049, #72117, #19293, #64945 ) ) ;
#33794=EDGE_CURVE ( 'NONE', #97645, #46755, #79034, .T. ) ;
#33795=CARTESIAN_POINT ( 'NONE',  ( -6.900000000000019007, 2.500000000000000000, -0.4464101615137783252 ) ) ;
#33796=DIRECTION ( 'NONE',  ( -0.000000000000000000, -1.000000000000000000, -0.000000000000000000 ) ) ;
#33798=ORIENTED_EDGE ( 'NONE', *, *, #38536, .F. ) ;
#33799=CIRCLE ( 'NONE', #75557, 0.1000000000000000472 ) ;
#33801=PLANE ( 'NONE',  #92842 ) ;
#33802=CARTESIAN_POINT ( 'NONE',  ( 13.29999999999990301, 12.50000000000000000, -4.330127018922201643 ) ) ;
#33803=CONICAL_SURFACE ( 'NONE', #109005, 0.1000000000000000472, 0.003490658503988666988 ) ;
#33804=CARTESIAN_POINT ( 'NONE',  ( -4.800000000000028244, 2.500000000000000000, -3.883716857408426648 ) ) ;
#33805=ORIENTED_EDGE ( 'NONE', *, *, #30758, .F. ) ;
#33806=AXIS2_PLACEMENT_3D ( 'NONE', #105622, #7394, #125255 ) ;
#33807=AXIS2_PLACEMENT_3D ( 'NONE', #10219, #51450, #30527 ) ;
#33808=ORIENTED_EDGE ( 'NONE', *, *, #21646, .T. ) ;
#33809=ORIENTED_EDGE ( 'NONE', *, *, #39436, .F. ) ;
#33810=ORIENTED_EDGE ( 'NONE', *, *, #69256, .F. ) ;
#33811=ORIENTED_EDGE ( 'NONE', *, *, #1527, .F. ) ;
#33812=CARTESIAN_POINT ( 'NONE',  ( -9.350000000000006750, 12.50000000000000000, 1.818653347947321475 ) ) ;
#33813=CARTESIAN_POINT ( 'NONE',  ( 11.64999999999990443, 2.500000000000000000, -7.288010851410854585 ) ) ;
#33814=VERTEX_POINT ( 'NONE', #49573 ) ;
#33815=FACE_BOUND ( 'NONE', #80859, .T. ) ;
#33816=CARTESIAN_POINT ( 'NONE',  ( 2.899999999999946620, 12.50000000000000000, -0.6928203230275542523 ) ) ;
#33817=ORIENTED_EDGE ( 'NONE', *, *, #57256, .T. ) ;
#33818=DIRECTION ( 'NONE',  ( -0.000000000000000000, 1.000000000000000000, -0.000000000000000000 ) ) ;
#33819=CARTESIAN_POINT ( 'NONE',  ( 2.299999999999949640, 12.50000000000000000, -4.676537180435977881 ) ) ;
#33820=FACE_OUTER_BOUND ( 'NONE', #100910, .T. ) ;
#33821=EDGE_LOOP ( 'NONE', ( #49057, #13272, #1917, #126046 ) ) ;
#33822=CARTESIAN_POINT ( 'NONE',  ( -11.05000000000000249, 12.50000000000000000, -1.818653347947322141 ) ) ;
#33823=EDGE_LOOP ( 'NONE', ( #60738, #79566 ) ) ;
#33824=ADVANCED_FACE ( 'NONE', ( #29928 ), #98699, .T. ) ;
#33825=ORIENTED_EDGE ( 'NONE', *, *, #121965, .F. ) ;
#33826=CIRCLE ( 'NONE', #81845, 0.1000000000000000472 ) ;
#33827=ORIENTED_EDGE ( 'NONE', *, *, #127498, .T. ) ;
#33828=VECTOR ( 'NONE', #39731, 1000.000000000000000 ) ;
#33829=CARTESIAN_POINT ( 'NONE',  ( -4.800000000000022915, 2.500000000000000000, 4.083716857408420609 ) ) ;
#33830=CARTESIAN_POINT ( 'NONE',  ( 5.849999999999933920, 2.500000000000000000, 6.595190528383296780 ) ) ;
#33831=CARTESIAN_POINT ( 'NONE',  ( -0.2000000000000339284, 2.500000000000000000, -0.2464101615137759549 ) ) ;
#33832=VERTEX_POINT ( 'NONE', #98005 ) ;
#33833=DIRECTION ( 'NONE',  ( 0.000000000000000000, 0.000000000000000000, -1.000000000000000000 ) ) ;
#33834=DIRECTION ( 'NONE',  ( 0.000000000000000000, 0.000000000000000000, 1.000000000000000000 ) ) ;
#33835=CIRCLE ( 'NONE', #58888, 0.1000000000000002554 ) ;
#33836=AXIS2_PLACEMENT_3D ( 'NONE', #17076, #57697, #124005 ) ;
#33837=CARTESIAN_POINT ( 'NONE',  ( -1.450000000000035927, 2.500000000000000000, -6.248780366869526759 ) ) ;
#33839=ORIENTED_EDGE ( 'NONE', *, *, #98433, .T. ) ;
#33840=AXIS2_PLACEMENT_3D ( 'NONE', #52048, #335, #101790 ) ;
#33841=AXIS2_PLACEMENT_3D ( 'NONE', #122638, #53898, #13308 ) ;
#33842=FACE_OUTER_BOUND ( 'NONE', #21141, .T. ) ;
#33843=ORIENTED_EDGE ( 'NONE', *, *, #37923, .F. ) ;
#33844=FACE_OUTER_BOUND ( 'NONE', #530, .T. ) ;
#33845=CONICAL_SURFACE ( 'NONE', #73541, 0.1000000000000002554, 0.003490658503988666988 ) ;
#33846=EDGE_LOOP ( 'NONE', ( #86977, #47355, #64084, #26060 ) ) ;
#33847=ORIENTED_EDGE ( 'NONE', *, *, #16615, .F. ) ;
#33848=CARTESIAN_POINT ( 'NONE',  ( 6.849999999999929479, 2.500000000000000000, 6.148780366869520009 ) ) ;
#33849=FACE_OUTER_BOUND ( 'NONE', #63865, .T. ) ;
#33850=FACE_OUTER_BOUND ( 'NONE', #62983, .T. ) ;
#33851=CARTESIAN_POINT ( 'NONE',  ( 3.299999999999944755, 12.50000000000000000, -4.330127018922201643 ) ) ;
#33852=DIRECTION ( 'NONE',  ( 0.000000000000000000, -0.9999939076577903929, 0.003490651415223739937 ) ) ;
#33853=ORIENTED_EDGE ( 'NONE', *, *, #77695, .F. ) ;
#33854=VERTEX_POINT ( 'NONE', #28640 ) ;
#33855=CARTESIAN_POINT ( 'NONE',  ( -6.250000000000017764, 2.500000000000000000, 2.857883832488649301 ) ) ;
#33857=DIRECTION ( 'NONE',  ( 0.000000000000000000, 0.000000000000000000, 1.000000000000000000 ) ) ;
#33858=ORIENTED_EDGE ( 'NONE', *, *, #20768, .F. ) ;
#33859=ORIENTED_EDGE ( 'NONE', *, *, #96525, .F. ) ;
#33860=DIRECTION ( 'NONE',  ( 0.000000000000000000, 0.000000000000000000, -1.000000000000000000 ) ) ;
#33861=VECTOR ( 'NONE', #51473, 1000.000000000000000 ) ;
#33862=ORIENTED_EDGE ( 'NONE', *, *, #23228, .T. ) ;
#33863=FACE_OUTER_BOUND ( 'NONE', #106769, .T. ) ;
#33864=AXIS2_PLACEMENT_3D ( 'NONE', #57058, #104866, #44684 ) ;
#33865=ADVANCED_FACE ( 'NONE', ( #117624 ), #69372, .T. ) ;
#33866=DIRECTION ( 'NONE',  ( 0.000000000000000000, 0.000000000000000000, 1.000000000000000000 ) ) ;
#33867=VERTEX_POINT ( 'NONE', #90104 ) ;
#33868=CARTESIAN_POINT ( 'NONE',  ( 10.79999999999991012, 12.50000000000000000, 4.330127018922196314 ) ) ;
#33869=DIRECTION ( 'NONE',  ( -0.000000000000000000, 1.000000000000000000, -0.000000000000000000 ) ) ;
#33870=DIRECTION ( 'NONE',  ( 0.000000000000000000, 1.000000000000000000, 0.000000000000000000 ) ) ;
#33871=EDGE_CURVE ( 'NONE', #56128, #47717, #15058, .T. ) ;
#33872=DIRECTION ( 'NONE',  ( 0.000000000000000000, 0.000000000000000000, 1.000000000000000000 ) ) ;
#33873=AXIS2_PLACEMENT_3D ( 'NONE', #60045, #39764, #108469 ) ;
#33874=EDGE_CURVE ( 'NONE', #117143, #79361, #99309, .T. ) ;
#33875=EDGE_LOOP ( 'NONE', ( #59175, #99892 ) ) ;
#33876=AXIS2_PLACEMENT_3D ( 'NONE', #84083, #54621, #55919 ) ;
#33877=CIRCLE ( 'NONE', #10865, 0.06509327318403745899 ) ;
#33878=CARTESIAN_POINT ( 'NONE',  ( 14.34999999999989306, 2.500000000000000000, -1.718653347947326049 ) ) ;
#33879=CONICAL_SURFACE ( 'NONE', #88228, 0.1000000000000002554, 0.003490658503988666988 ) ;
#33880=CARTESIAN_POINT ( 'NONE',  ( 32.27111852103835332, -3.178312372601638902, 3.140919221367066694 ) ) ;
#33881=ADVANCED_FACE ( 'NONE', ( #434 ), #127481, .T. ) ;
#33882=VERTEX_POINT ( 'NONE', #29284 ) ;
#33883=EDGE_CURVE ( 'NONE', #47772, #21032, #406, .T. ) ;
#33884=ORIENTED_EDGE ( 'NONE', *, *, #62875, .T. ) ;
#33885=ADVANCED_FACE ( 'NONE', ( #116988 ), #109064, .T. ) ;
#33887=DIRECTION ( 'NONE',  ( 0.000000000000000000, 0.000000000000000000, -1.000000000000000000 ) ) ;
#33888=EDGE_CURVE ( 'NONE', #96407, #35702, #50597, .T. ) ;
#33889=ADVANCED_FACE ( 'NONE', ( #39125 ), #115322, .T. ) ;
#33890=DIRECTION ( 'NONE',  ( 0.000000000000000000, 0.000000000000000000, -1.000000000000000000 ) ) ;
#33891=AXIS2_PLACEMENT_3D ( 'NONE', #5273, #125687, #16367 ) ;
#33892=DIRECTION ( 'NONE',  ( -0.000000000000000000, -1.000000000000000000, -0.000000000000000000 ) ) ;
#33893=DIRECTION ( 'NONE',  ( -0.000000000000000000, -1.000000000000000000, -0.000000000000000000 ) ) ;
#33894=AXIS2_PLACEMENT_3D ( 'NONE', #74052, #72764, #113977 ) ;
#33895=DIRECTION ( 'NONE',  ( -0.000000000000000000, -1.000000000000000000, -0.000000000000000000 ) ) ;
#33896=CARTESIAN_POINT ( 'NONE',  ( 9.399999999999918643, 2.500000000000000000, 0.3464101615137736845 ) ) ;
#33897=CONICAL_SURFACE ( 'NONE', #107033, 0.09999999999999982514, 0.003490658503988666988 ) ;
#33898=CARTESIAN_POINT ( 'NONE',  ( 1.249999999999950262, 12.50000000000000000, 7.253104124594885960 ) ) ;
#33899=AXIS2_PLACEMENT_3D ( 'NONE', #40819, #80731, #121288 ) ;
#33901=VECTOR ( 'NONE', #74096, 1000.000000000000000 ) ;
#33902=CARTESIAN_POINT ( 'NONE',  ( 4.199999999999939782, 12.50000000000000000, -0.06509327318403970719 ) ) ;
#33903=ADVANCED_FACE ( 'NONE', ( #107179 ), #69845, .T. ) ;
#33904=CARTESIAN_POINT ( 'NONE',  ( 13.54999999999989591, 2.500000000000000000, -1.818653347947326138 ) ) ;
#33905=ORIENTED_EDGE ( 'NONE', *, *, #83952, .F. ) ;
#33906=EDGE_CURVE ( 'NONE', #51386, #44872, #12927, .T. ) ;
#33907=ORIENTED_EDGE ( 'NONE', *, *, #322, .F. ) ;
#33908=CONICAL_SURFACE ( 'NONE', #54723, 0.1000000000000002554, 0.003490658503988666988 ) ;
#33909=ORIENTED_EDGE ( 'NONE', *, *, #37309, .F. ) ;
#33910=EDGE_LOOP ( 'NONE', ( #80048, #3964, #64613, #38394 ) ) ;
#33911=DIRECTION ( 'NONE',  ( -0.000000000000000000, -1.000000000000000000, -0.000000000000000000 ) ) ;
#33912=CARTESIAN_POINT ( 'NONE',  ( -3.350000000000028511, 12.50000000000000000, -1.537336459617587581 ) ) ;
#33913=ORIENTED_EDGE ( 'NONE', *, *, #19009, .T. ) ;
#33914=CARTESIAN_POINT ( 'NONE',  ( -3.350000000000028511, 2.500000000000000000, -2.757883832488654097 ) ) ;
#33915=PLANE ( 'NONE',  #5415 ) ;
#33916=DIRECTION ( 'NONE',  ( 0.000000000000000000, 0.000000000000000000, 1.000000000000000000 ) ) ;
#33917=VERTEX_POINT ( 'NONE', #87539 ) ;
#33918=DIRECTION ( 'NONE',  ( 0.000000000000000000, 0.000000000000000000, 1.000000000000000000 ) ) ;
#33919=DIRECTION ( 'NONE',  ( -4.274815082592931898E-19, -0.9999939076577903929, -0.003490651415223739937 ) ) ;
#33920=EDGE_LOOP ( 'NONE', ( #54497, #39197, #54856, #27292 ) ) ;
#33921=ORIENTED_EDGE ( 'NONE', *, *, #122605, .F. ) ;
#33923=VECTOR ( 'NONE', #3063, 1000.000000000000000 ) ;
#33924=VERTEX_POINT ( 'NONE', #67903 ) ;
#33925=DIRECTION ( 'NONE',  ( 0.000000000000000000, 0.000000000000000000, -1.000000000000000000 ) ) ;
#33926=AXIS2_PLACEMENT_3D ( 'NONE', #55828, #65643, #16525 ) ;
#33927=CIRCLE ( 'NONE', #27639, 0.06509327318403741736 ) ;
#33930=DIRECTION ( 'NONE',  ( -0.000000000000000000, -1.000000000000000000, -0.000000000000000000 ) ) ;
#33931=CARTESIAN_POINT ( 'NONE',  ( 13.34999999999989662, 12.50000000000000000, -2.099970236277064473 ) ) ;
#33932=EDGE_CURVE ( 'NONE', #76503, #37568, #29679, .T. ) ;
#33933=DIRECTION ( 'NONE',  ( 0.000000000000000000, 0.000000000000000000, -1.000000000000000000 ) ) ;
#33934=CONICAL_SURFACE ( 'NONE', #88185, 0.1000000000000002554, 0.003490658503988666988 ) ;
#33935=EDGE_LOOP ( 'NONE', ( #59005, #47633 ) ) ;
#33936=AXIS2_PLACEMENT_3D ( 'NONE', #42618, #94266, #43902 ) ;
#33937=EDGE_CURVE ( 'NONE', #124362, #127904, #88486, .T. ) ;
#33938=AXIS2_PLACEMENT_3D ( 'NONE', #100812, #109359, #39994 ) ;
#33939=DIRECTION ( 'NONE',  ( 0.000000000000000000, 0.000000000000000000, 1.000000000000000000 ) ) ;
#33940=CIRCLE ( 'NONE', #12982, 0.06509327318403743123 ) ;
#33941=ORIENTED_EDGE ( 'NONE', *, *, #46970, .T. ) ;
#33942=CARTESIAN_POINT ( 'NONE',  ( 9.549999999999918998, 12.50000000000000000, -6.430097255199264339 ) ) ;
#33943=CARTESIAN_POINT ( 'NONE',  ( 10.87377556642347010, -1.500000000000192513, -8.986829606637039447 ) ) ;
#33944=CIRCLE ( 'NONE', #46447, 0.1000000000000002554 ) ;
#33945=CARTESIAN_POINT ( 'NONE',  ( 11.64999999999990266, 12.50000000000000000, 2.099970236277060032 ) ) ;
#33946=CARTESIAN_POINT ( 'NONE',  ( -1.250000000000037526, 12.50000000000000000, -5.802370205355749988 ) ) ;
#33947=EDGE_CURVE ( 'NONE', #460, #25156, #100756, .T. ) ;
#33948=AXIS2_PLACEMENT_3D ( 'NONE', #53544, #92828, #50976 ) ;
#33950=EDGE_LOOP ( 'NONE', ( #68110, #38341 ) ) ;
#33951=EDGE_CURVE ( 'NONE', #54777, #109103, #102814, .T. ) ;
#33952=ORIENTED_EDGE ( 'NONE', *, *, #111281, .F. ) ;
#33953=ORIENTED_EDGE ( 'NONE', *, *, #97437, .T. ) ;
#33954=DIRECTION ( 'NONE',  ( -0.000000000000000000, -1.000000000000000000, -0.000000000000000000 ) ) ;
#33955=DIRECTION ( 'NONE',  ( 0.000000000000000000, 0.000000000000000000, 1.000000000000000000 ) ) ;
#33956=DIRECTION ( 'NONE',  ( 0.000000000000000000, 1.000000000000000000, 0.000000000000000000 ) ) ;
#33957=FACE_BOUND ( 'NONE', #116548, .T. ) ;
#33958=LINE ( 'NONE', #22222, #116171 ) ;
#33959=CARTESIAN_POINT ( 'NONE',  ( 5.199999999999935341, 2.500000000000000000, -3.883716857408426648 ) ) ;
#33960=EDGE_CURVE ( 'NONE', #128018, #92934, #46381, .T. ) ;
#33961=CARTESIAN_POINT ( 'NONE',  ( 5.849999999999932143, 2.500000000000000000, 1.472243186433545459 ) ) ;
#33962=CIRCLE ( 'NONE', #113655, 0.1000000000000002554 ) ;
#33963=CARTESIAN_POINT ( 'NONE',  ( -9.400000000000009237, 2.500000000000000000, -3.983716857408421852 ) ) ;
#33964=CARTESIAN_POINT ( 'NONE',  ( -11.24999999999996447, 12.50000000000000000, -2.165063509461097713 ) ) ;
#33965=DIRECTION ( 'NONE',  ( -0.000000000000000000, 1.000000000000000000, -0.000000000000000000 ) ) ;
#33967=AXIS2_PLACEMENT_3D ( 'NONE', #37636, #97822, #105722 ) ;
#33968=CONICAL_SURFACE ( 'NONE', #73960, 0.09999999999999999167, 0.003490658503988666988 ) ;
#33969=CARTESIAN_POINT ( 'NONE',  ( 10.84999999999991260, 2.500000000000000000, -2.065063509461102065 ) ) ;
#33970=VERTEX_POINT ( 'NONE', #1731 ) ;
#33971=EDGE_LOOP ( 'NONE', ( #9444, #67582, #56358, #31533 ) ) ;
#33973=VERTEX_POINT ( 'NONE', #41691 ) ;
#33974=CARTESIAN_POINT ( 'NONE',  ( 9.149999999999918643, 12.50000000000000000, 2.099970236277060032 ) ) ;
#33975=EDGE_CURVE ( 'NONE', #122222, #83264, #63243, .T. ) ;
#33976=FACE_BOUND ( 'NONE', #26646, .T. ) ;
#33977=AXIS2_PLACEMENT_3D ( 'NONE', #103818, #6230, #113635 ) ;
#33978=DIRECTION ( 'NONE',  ( 0.000000000000000000, 1.000000000000000000, 0.000000000000000000 ) ) ;
#33979=CIRCLE ( 'NONE', #90386, 0.1000000000000002554 ) ;
#33980=ORIENTED_EDGE ( 'NONE', *, *, #47504, .F. ) ;
#33981=CARTESIAN_POINT ( 'NONE',  ( 21.23528140090950700, 2.699413673072311060, 2.293764360948887138 ) ) ;
#33982=CARTESIAN_POINT ( 'NONE',  ( -2.900000000000029221, 2.500000000000000000, -4.230127018922201998 ) ) ;
#33983=ORIENTED_EDGE ( 'NONE', *, *, #42167, .F. ) ;
#33984=CIRCLE ( 'NONE', #75826, 0.1000000000000000472 ) ;
#33985=DIRECTION ( 'NONE',  ( 0.000000000000000000, 0.000000000000000000, -1.000000000000000000 ) ) ;
#33986=FACE_OUTER_BOUND ( 'NONE', #126921, .T. ) ;
#33987=CONICAL_SURFACE ( 'NONE', #125998, 0.1000000000000000472, 0.003490658503988666988 ) ;
#33988=ADVANCED_FACE ( 'NONE', ( #31857 ), #73571, .T. ) ;
#33989=AXIS2_PLACEMENT_3D ( 'NONE', #34033, #4535, #13730 ) ;
#33990=AXIS2_PLACEMENT_3D ( 'NONE', #25489, #54325, #115141 ) ;
#33991=AXIS2_PLACEMENT_3D ( 'NONE', #35312, #83755, #115116 ) ;
#33992=EDGE_LOOP ( 'NONE', ( #68376, #128564, #77335, #65646 ) ) ;
#33993=DIRECTION ( 'NONE',  ( 0.000000000000000000, 1.000000000000000000, 0.000000000000000000 ) ) ;
#33994=CARTESIAN_POINT ( 'NONE',  ( 10.39999999999990976, 12.50000000000000000, 4.330127018922196314 ) ) ;
#33995=VECTOR ( 'NONE', #95468, 1000.000000000000000 ) ;
#33996=ORIENTED_EDGE ( 'NONE', *, *, #37368, .F. ) ;
#33997=DIRECTION ( 'NONE',  ( 0.000000000000000000, 0.000000000000000000, -1.000000000000000000 ) ) ;
#33998=CONICAL_SURFACE ( 'NONE', #75750, 0.09999999999999982514, 0.003490658503988666988 ) ;
#34000=DIRECTION ( 'NONE',  ( 0.000000000000000000, 0.000000000000000000, -1.000000000000000000 ) ) ;
#34001=ORIENTED_EDGE ( 'NONE', *, *, #61518, .F. ) ;
#34002=ORIENTED_EDGE ( 'NONE', *, *, #61515, .T. ) ;
#34003=EDGE_CURVE ( 'NONE', #125076, #885, #56831, .T. ) ;
#34004=CARTESIAN_POINT ( 'NONE',  ( -0.6000000000000388356, 2.500000000000000000, 4.776537180435972196 ) ) ;
#34005=ORIENTED_EDGE ( 'NONE', *, *, #123477, .F. ) ;
#34006=DIRECTION ( 'NONE',  ( 0.000000000000000000, 1.000000000000000000, 0.000000000000000000 ) ) ;
#34007=DIRECTION ( 'NONE',  ( 0.000000000000000000, 0.000000000000000000, 1.000000000000000000 ) ) ;
#34008=EDGE_LOOP ( 'NONE', ( #80612, #124042 ) ) ;
#34009=DIRECTION ( 'NONE',  ( 0.000000000000000000, 0.000000000000000000, -1.000000000000000000 ) ) ;
#34010=CARTESIAN_POINT ( 'NONE',  ( -4.999999999999986677, 2.500000000000000000, 4.330127018922196314 ) ) ;
#34011=DIRECTION ( 'NONE',  ( 0.000000000000000000, 1.000000000000000000, 0.000000000000000000 ) ) ;
#34012=DIRECTION ( 'NONE',  ( -0.000000000000000000, -1.000000000000000000, -0.000000000000000000 ) ) ;
#34013=AXIS2_PLACEMENT_3D ( 'NONE', #17790, #59021, #57743 ) ;
#34014=CARTESIAN_POINT ( 'NONE',  ( -3.749999999999991562, 12.50000000000000000, 6.495190528383297135 ) ) ;
#34015=VERTEX_POINT ( 'NONE', #22693 ) ;
#34016=ORIENTED_EDGE ( 'NONE', *, *, #101145, .T. ) ;
#34017=CARTESIAN_POINT ( 'NONE',  ( 9.199999999999915801, 12.50000000000000000, -4.330127018922201643 ) ) ;
#34018=CONICAL_SURFACE ( 'NONE', #19330, 0.1000000000000002554, 0.003490658503988666988 ) ;
#34020=CONICAL_SURFACE ( 'NONE', #90426, 0.1000000000000002554, 0.003490658503988666988 ) ;
#34021=ORIENTED_EDGE ( 'NONE', *, *, #100245, .F. ) ;
#34022=EDGE_LOOP ( 'NONE', ( #34184, #124683 ) ) ;
#34023=ORIENTED_EDGE ( 'NONE', *, *, #1160, .T. ) ;
#34024=DIRECTION ( 'NONE',  ( -0.000000000000000000, 1.000000000000000000, -0.000000000000000000 ) ) ;
#34025=DIRECTION ( 'NONE',  ( 0.000000000000000000, 1.000000000000000000, 0.000000000000000000 ) ) ;
#34026=AXIS2_PLACEMENT_3D ( 'NONE', #102768, #81221, #13093 ) ;
#34027=AXIS2_PLACEMENT_3D ( 'NONE', #69979, #79789, #78528 ) ;
#34028=CARTESIAN_POINT ( 'NONE',  ( -6.700000000000019718, 12.50000000000000000, -4.330127018922201643 ) ) ;
#34029=EDGE_CURVE ( 'NONE', #27373, #57931, #90764, .T. ) ;
#34031=LINE ( 'NONE', #113219, #39001 ) ;
#34032=CARTESIAN_POINT ( 'NONE',  ( -13.09999999999999254, 2.500000000000000000, 0.3464101615137777923 ) ) ;
#34033=CARTESIAN_POINT ( 'NONE',  ( 12.89999999999990266, 12.50000000000000000, -5.022947341949754119 ) ) ;
#34034=DIRECTION ( 'NONE',  ( 0.000000000000000000, 0.000000000000000000, 1.000000000000000000 ) ) ;
#34035=DIRECTION ( 'NONE',  ( -0.000000000000000000, 1.000000000000000000, -0.000000000000000000 ) ) ;
#34036=AXIS2_PLACEMENT_3D ( 'NONE', #79530, #119433, #295 ) ;
#34037=CIRCLE ( 'NONE', #57303, 0.06509327318403745899 ) ;
#34038=LINE ( 'NONE', #125620, #129319 ) ;
#34039=EDGE_CURVE ( 'NONE', #98092, #63695, #19280, .T. ) ;
#34040=ORIENTED_EDGE ( 'NONE', *, *, #41972, .T. ) ;
#34041=CARTESIAN_POINT ( 'NONE',  ( -5.450000000000019718, 2.500000000000000000, 6.495190528383297135 ) ) ;
#34042=EDGE_CURVE ( 'NONE', #41518, #10631, #79935, .T. ) ;
#34043=ORIENTED_EDGE ( 'NONE', *, *, #66010, .F. ) ;
#34044=EDGE_CURVE ( 'NONE', #62494, #117214, #123442, .T. ) ;
#34045=ORIENTED_EDGE ( 'NONE', *, *, #6599, .T. ) ;
#34046=ADVANCED_FACE ( 'NONE', ( #54068 ), #95285, .T. ) ;
#34047=CARTESIAN_POINT ( 'NONE',  ( -8.550000000000013145, 2.500000000000000000, -1.818653347947326138 ) ) ;
#34048=CARTESIAN_POINT ( 'NONE',  ( 6.649999999999928413, 2.500000000000000000, 1.472243186433545459 ) ) ;
#34049=ADVANCED_FACE ( 'NONE', ( #46178 ), #75619, .T. ) ;
#34050=DIRECTION ( 'NONE',  ( 0.000000000000000000, 0.000000000000000000, -1.000000000000000000 ) ) ;
#34051=CIRCLE ( 'NONE', #69537, 0.1000000000000002554 ) ;
#34052=CARTESIAN_POINT ( 'NONE',  ( -6.450000000000016165, 12.50000000000000000, 2.511473670974873507 ) ) ;
#34053=DIRECTION ( 'NONE',  ( 0.000000000000000000, 0.000000000000000000, -1.000000000000000000 ) ) ;
#34054=ADVANCED_FACE ( 'NONE', ( #55987 ), #92456, .T. ) ;
#34055=CARTESIAN_POINT ( 'NONE',  ( -11.64999999999999680, 12.50000000000000000, 1.472243186433545459 ) ) ;
#34056=DIRECTION ( 'NONE',  ( -0.000000000000000000, -1.000000000000000000, -0.000000000000000000 ) ) ;
#34057=VERTEX_POINT ( 'NONE', #14754 ) ;
#34059=EDGE_CURVE ( 'NONE', #18421, #68242, #121782, .T. ) ;
#34060=AXIS2_PLACEMENT_3D ( 'NONE', #91880, #2192, #74174 ) ;
#34061=CARTESIAN_POINT ( 'NONE',  ( -7.500000000000015099, 2.500000000000000000, -0.6928203230275541413 ) ) ;
#34062=CONICAL_SURFACE ( 'NONE', #98792, 0.1000000000000002554, 0.003490658503988666988 ) ;
#34064=VERTEX_POINT ( 'NONE', #24612 ) ;
#34065=CIRCLE ( 'NONE', #82079, 0.06509327318403745899 ) ;
#34066=EDGE_CURVE ( 'NONE', #123447, #10798, #36028, .T. ) ;
#34067=EDGE_LOOP ( 'NONE', ( #25216, #95832 ) ) ;
#34068=ORIENTED_EDGE ( 'NONE', *, *, #58639, .T. ) ;
#34069=EDGE_LOOP ( 'NONE', ( #73043, #125853, #124220, #6470 ) ) ;
#34070=AXIS2_PLACEMENT_3D ( 'NONE', #89962, #40229, #282 ) ;
#34071=ADVANCED_FACE ( 'NONE', ( #105082 ), #86173, .T. ) ;
#34072=CARTESIAN_POINT ( 'NONE',  ( 2.299999999999949640, 2.500000000000000000, -0.4464101615137782142 ) ) ;
#34073=CARTESIAN_POINT ( 'NONE',  ( 6.899999999999928413, 2.500000000000000000, 4.776537180435972196 ) ) ;
#34074=VECTOR ( 'NONE', #28088, 1000.000000000000000 ) ;
#34075=AXIS2_PLACEMENT_3D ( 'NONE', #19011, #31439, #58328 ) ;
#34076=CARTESIAN_POINT ( 'NONE',  ( -2.050000000000032685, 2.500000000000000000, -6.595190528383302109 ) ) ;
#34077=DIRECTION ( 'NONE',  ( 0.000000000000000000, 0.000000000000000000, -1.000000000000000000 ) ) ;
#34078=DIRECTION ( 'NONE',  ( -0.000000000000000000, 1.000000000000000000, -0.000000000000000000 ) ) ;
#34079=VERTEX_POINT ( 'NONE', #124093 ) ;
#34080=DIRECTION ( 'NONE',  ( 0.000000000000000000, -0.9999939076577903929, 0.003490651415223739937 ) ) ;
#34081=DIRECTION ( 'NONE',  ( -4.274815082592931898E-19, -0.9999939076577903929, -0.003490651415223739937 ) ) ;
#34082=AXIS2_PLACEMENT_3D ( 'NONE', #104615, #84341, #77103 ) ;
#34083=AXIS2_PLACEMENT_3D ( 'NONE', #91379, #1701, #81563 ) ;
#34084=CARTESIAN_POINT ( 'NONE',  ( -4.150000000000028777, 2.500000000000000000, -5.802370205355749988 ) ) ;
#34085=ORIENTED_EDGE ( 'NONE', *, *, #126087, .T. ) ;
#34086=CIRCLE ( 'NONE', #21560, 0.06509327318403743123 ) ;
#34087=CONICAL_SURFACE ( 'NONE', #121806, 0.09999999999999982514, 0.003490658503988666988 ) ;
#34088=CONICAL_SURFACE ( 'NONE', #23716, 0.09999999999999982514, 0.003490658503988666988 ) ;
#34089=VERTEX_POINT ( 'NONE', #55359 ) ;
#34090=ORIENTED_EDGE ( 'NONE', *, *, #123160, .F. ) ;
#34091=FACE_OUTER_BOUND ( 'NONE', #2039, .T. ) ;
#34092=CONICAL_SURFACE ( 'NONE', #69587, 0.1000000000000002554, 0.003490658503988666988 ) ;
#34093=DIRECTION ( 'NONE',  ( -0.000000000000000000, -1.000000000000000000, -0.000000000000000000 ) ) ;
#34095=AXIS2_PLACEMENT_3D ( 'NONE', #56819, #58154, #98057 ) ;
#34096=EDGE_LOOP ( 'NONE', ( #55695, #93011, #95463, #104196 ) ) ;
#34097=DIRECTION ( 'NONE',  ( 0.000000000000000000, 0.000000000000000000, 1.000000000000000000 ) ) ;
#34098=DIRECTION ( 'NONE',  ( -0.000000000000000000, -1.000000000000000000, -0.000000000000000000 ) ) ;
#34099=CARTESIAN_POINT ( 'NONE',  ( 2.949999999999945111, 12.50000000000000000, 2.165063509461097713 ) ) ;
#34100=DIRECTION ( 'NONE',  ( -0.000000000000000000, -1.000000000000000000, -0.000000000000000000 ) ) ;
#34101=EDGE_CURVE ( 'NONE', #65379, #126646, #48644, .T. ) ;
#34102=CARTESIAN_POINT ( 'NONE',  ( -14.59999999999998366, 2.500000000000000000, -0.6928203230275520319 ) ) ;
#34103=EDGE_CURVE ( 'NONE', #99278, #90531, #116196, .T. ) ;
#34104=ORIENTED_EDGE ( 'NONE', *, *, #12811, .T. ) ;
#34105=CONICAL_SURFACE ( 'NONE', #107255, 0.1000000000000002554, 0.003490658503988666988 ) ;
#34106=ORIENTED_EDGE ( 'NONE', *, *, #24167, .F. ) ;
#34107=CONICAL_SURFACE ( 'NONE', #67528, 0.09999999999999982514, 0.003490658503988666988 ) ;
#34109=FACE_OUTER_BOUND ( 'NONE', #31887, .T. ) ;
#34110=DIRECTION ( 'NONE',  ( -0.000000000000000000, 1.000000000000000000, -0.000000000000000000 ) ) ;
#34111=DIRECTION ( 'NONE',  ( -0.000000000000000000, -1.000000000000000000, -0.000000000000000000 ) ) ;
#34112=EDGE_CURVE ( 'NONE', #76479, #16894, #56926, .T. ) ;
#34113=DIRECTION ( 'NONE',  ( 0.000000000000000000, 1.000000000000000000, 0.000000000000000000 ) ) ;
#34114=ORIENTED_EDGE ( 'NONE', *, *, #65949, .T. ) ;
#34115=AXIS2_PLACEMENT_3D ( 'NONE', #64509, #94611, #24595 ) ;
#34116=CIRCLE ( 'NONE', #73811, 0.06509327318403745899 ) ;
#34117=AXIS2_PLACEMENT_3D ( 'NONE', #122249, #120940, #32596 ) ;
#34118=AXIS2_PLACEMENT_3D ( 'NONE', #56574, #93947, #106339 ) ;
#34119=ORIENTED_EDGE ( 'NONE', *, *, #76568, .F. ) ;
#34120=DIRECTION ( 'NONE',  ( 0.000000000000000000, 0.000000000000000000, -1.000000000000000000 ) ) ;
#34121=CARTESIAN_POINT ( 'NONE',  ( 1.699999999999950218, 12.50000000000000000, 4.330127018922196314 ) ) ;
#34122=CARTESIAN_POINT ( 'NONE',  ( 17.50982738792208693, -2.500000000000000000, -4.074750937467086054 ) ) ;
#34123=CARTESIAN_POINT ( 'NONE',  ( -9.400000000000007461, 2.500000000000000000, 0.3464101615137735735 ) ) ;
#34124=VERTEX_POINT ( 'NONE', #45550 ) ;
#34125=CIRCLE ( 'NONE', #40391, 0.06509327318403741736 ) ;
#34126=LINE ( 'NONE', #15747, #78286 ) ;
#34127=AXIS2_PLACEMENT_3D ( 'NONE', #107149, #94764, #76422 ) ;
#34128=CIRCLE ( 'NONE', #15317, 0.06509327318403745899 ) ;
#34129=CARTESIAN_POINT ( 'NONE',  ( 1.249999999999952482, 2.500000000000000000, -5.902370205355750521 ) ) ;
#34130=CONICAL_SURFACE ( 'NONE', #78032, 0.1000000000000002554, 0.003490658503988666988 ) ;
#34132=DIRECTION ( 'NONE',  ( 0.000000000000000000, 0.000000000000000000, -1.000000000000000000 ) ) ;
#34133=ORIENTED_EDGE ( 'NONE', *, *, #7482, .F. ) ;
#34134=CIRCLE ( 'NONE', #96810, 0.1000000000000000472 ) ;
#34135=LINE ( 'NONE', #113974, #49301 ) ;
#34136=ORIENTED_EDGE ( 'NONE', *, *, #12413, .F. ) ;
#34137=DIRECTION ( 'NONE',  ( 0.000000000000000000, 0.000000000000000000, 1.000000000000000000 ) ) ;
#34138=CARTESIAN_POINT ( 'NONE',  ( 9.349999999999919709, 12.50000000000000000, 2.576566944158910744 ) ) ;
#34139=ORIENTED_EDGE ( 'NONE', *, *, #106779, .T. ) ;
#34140=ORIENTED_EDGE ( 'NONE', *, *, #96858, .F. ) ;
#34142=CARTESIAN_POINT ( 'NONE',  ( -9.150000000000005684, 2.500000000000000000, 5.802370205355744659 ) ) ;
#34145=DIRECTION ( 'NONE',  ( 0.000000000000000000, 1.000000000000000000, 0.000000000000000000 ) ) ;
#34146=DIRECTION ( 'NONE',  ( 0.000000000000000000, 1.000000000000000000, 0.000000000000000000 ) ) ;
#34147=CARTESIAN_POINT ( 'NONE',  ( 10.79999999999991367, 2.500000000000000000, -2.385244779468109755E-15 ) ) ;
#34148=DIRECTION ( 'NONE',  ( -0.000000000000000000, -1.000000000000000000, -0.000000000000000000 ) ) ;
#34149=CONICAL_SURFACE ( 'NONE', #126073, 0.1000000000000002554, 0.003490658503988666988 ) ;
#34150=AXIS2_PLACEMENT_3D ( 'NONE', #75492, #113493, #23841 ) ;
#34151=AXIS2_PLACEMENT_3D ( 'NONE', #28196, #27525, #18997 ) ;
#34153=ORIENTED_EDGE ( 'NONE', *, *, #109904, .F. ) ;
#34154=DIRECTION ( 'NONE',  ( -0.000000000000000000, -1.000000000000000000, -0.000000000000000000 ) ) ;
#34155=CARTESIAN_POINT ( 'NONE',  ( -1.050000000000037792, 2.500000000000000000, 6.048780366869520364 ) ) ;
#34156=DIRECTION ( 'NONE',  ( 0.000000000000000000, -0.9999939076577903929, 0.003490651415223739937 ) ) ;
#34157=EDGE_CURVE ( 'NONE', #124875, #8330, #65347, .T. ) ;
#34158=DIRECTION ( 'NONE',  ( 0.000000000000000000, 0.000000000000000000, 1.000000000000000000 ) ) ;
#34159=ORIENTED_EDGE ( 'NONE', *, *, #105596, .T. ) ;
#34160=ORIENTED_EDGE ( 'NONE', *, *, #65210, .T. ) ;
#34161=FACE_BOUND ( 'NONE', #49684, .T. ) ;
#34162=EDGE_LOOP ( 'NONE', ( #54645, #105797 ) ) ;
#34163=EDGE_CURVE ( 'NONE', #100499, #41901, #115541, .T. ) ;
#34164=AXIS2_PLACEMENT_3D ( 'NONE', #81758, #121684, #32049 ) ;
#34165=CARTESIAN_POINT ( 'NONE',  ( 0.4499999999999573785, 2.500000000000000000, -6.595190528383302109 ) ) ;
#34166=CARTESIAN_POINT ( 'NONE',  ( 19.95908882845278853, -2.629614671951212568, 2.273431397254419117 ) ) ;
#34167=CIRCLE ( 'NONE', #67586, 0.06509327318403741736 ) ;
#34168=VERTEX_POINT ( 'NONE', #16052 ) ;
#34169=CIRCLE ( 'NONE', #29967, 0.1000000000000000472 ) ;
#34170=DIRECTION ( 'NONE',  ( -4.274815082592931898E-19, -0.9999939076577903929, -0.003490651415223739937 ) ) ;
#34171=DIRECTION ( 'NONE',  ( 0.000000000000000000, 1.000000000000000000, 0.000000000000000000 ) ) ;
#34172=CONICAL_SURFACE ( 'NONE', #126089, 0.1000000000000002554, 0.003490658503988666988 ) ;
#34173=DIRECTION ( 'NONE',  ( 0.000000000000000000, 1.000000000000000000, 0.000000000000000000 ) ) ;
#34174=FACE_OUTER_BOUND ( 'NONE', #6721, .T. ) ;
#34175=CARTESIAN_POINT ( 'NONE',  ( 6.049999999999934097, 12.50000000000000000, -6.083687093685488989 ) ) ;
#34176=DIRECTION ( 'NONE',  ( -0.000000000000000000, -1.000000000000000000, -0.000000000000000000 ) ) ;
#34177=EDGE_CURVE ( 'NONE', #70324, #104908, #66456, .T. ) ;
#34178=FACE_OUTER_BOUND ( 'NONE', #51136, .T. ) ;
#34179=DIRECTION ( 'NONE',  ( 0.000000000000000000, -0.9999939076577903929, 0.003490651415223739937 ) ) ;
#34180=AXIS2_PLACEMENT_3D ( 'NONE', #19000, #69397, #28199 ) ;
#34181=DIRECTION ( 'NONE',  ( 0.000000000000000000, 0.000000000000000000, -1.000000000000000000 ) ) ;
#34182=VERTEX_POINT ( 'NONE', #14125 ) ;
#34183=ORIENTED_EDGE ( 'NONE', *, *, #85471, .F. ) ;
#34184=ORIENTED_EDGE ( 'NONE', *, *, #80140, .T. ) ;
#34185=CARTESIAN_POINT ( 'NONE',  ( 11.04999999999991012, 12.50000000000000000, 6.841600689897072485 ) ) ;
#34186=AXIS2_PLACEMENT_3D ( 'NONE', #108311, #78231, #945 ) ;
#34187=ORIENTED_EDGE ( 'NONE', *, *, #115542, .T. ) ;
#34188=AXIS2_PLACEMENT_3D ( 'NONE', #118078, #107623, #49372 ) ;
#34189=CIRCLE ( 'NONE', #117768, 0.09999999999999982514 ) ;
#34190=ORIENTED_EDGE ( 'NONE', *, *, #9310, .F. ) ;
#34191=ORIENTED_EDGE ( 'NONE', *, *, #125283, .T. ) ;
#34192=VERTEX_POINT ( 'NONE', #84160 ) ;
#34193=AXIS2_PLACEMENT_3D ( 'NONE', #20630, #77590, #49460 ) ;
#34194=DIRECTION ( 'NONE',  ( 0.000000000000000000, -0.000000000000000000, 1.000000000000000000 ) ) ;
#34195=LINE ( 'NONE', #91815, #107364 ) ;
#34196=EDGE_CURVE ( 'NONE', #24753, #26449, #25900, .T. ) ;
#34198=FACE_OUTER_BOUND ( 'NONE', #30082, .T. ) ;
#34199=CARTESIAN_POINT ( 'NONE',  ( 6.849999999999930367, 12.50000000000000000, -6.148780366869526226 ) ) ;
#34200=DIRECTION ( 'NONE',  ( 0.000000000000000000, -0.9999939076577903929, 0.003490651415223739937 ) ) ;
#34201=ORIENTED_EDGE ( 'NONE', *, *, #98229, .T. ) ;
#34202=CARTESIAN_POINT ( 'NONE',  ( 12.04999999999990479, 2.500000000000000000, -6.495190528383302464 ) ) ;
#34203=VERTEX_POINT ( 'NONE', #74350 ) ;
#34204=EDGE_CURVE ( 'NONE', #117086, #103811, #114270, .T. ) ;
#34207=DIRECTION ( 'NONE',  ( 0.000000000000000000, 0.000000000000000000, -1.000000000000000000 ) ) ;
#34208=CONICAL_SURFACE ( 'NONE', #61391, 0.1000000000000002554, 0.003490658503988666988 ) ;
#34209=EDGE_CURVE ( 'NONE', #28566, #36792, #25644, .T. ) ;
#34210=CIRCLE ( 'NONE', #113611, 0.09999999999999982514 ) ;
#34211=EDGE_LOOP ( 'NONE', ( #3726, #53333, #92426, #107596 ) ) ;
#34212=ADVANCED_FACE ( 'NONE', ( #116838 ), #88009, .T. ) ;
#34213=ORIENTED_EDGE ( 'NONE', *, *, #116734, .T. ) ;
#34214=ADVANCED_FACE ( 'NONE', ( #109622 ), #42386, .T. ) ;
#34215=ORIENTED_EDGE ( 'NONE', *, *, #47711, .F. ) ;
#34216=ADVANCED_FACE ( 'NONE', ( #68390 ), #61159, .T. ) ;
#34217=DIRECTION ( 'NONE',  ( 0.000000000000000000, 1.000000000000000000, 0.000000000000000000 ) ) ;
#34218=CONICAL_SURFACE ( 'NONE', #15392, 0.09999999999999999167, 0.003490658503988666988 ) ;
#34219=CARTESIAN_POINT ( 'NONE',  ( -2.900000000000030553, 2.500000000000000000, 5.022947341949748790 ) ) ;
#34220=CONICAL_SURFACE ( 'NONE', #15393, 0.1000000000000002554, 0.003490658503988666988 ) ;
#34221=LINE ( 'NONE', #83317, #70935 ) ;
#34222=DIRECTION ( 'NONE',  ( 0.000000000000000000, 0.000000000000000000, 1.000000000000000000 ) ) ;
#34223=CARTESIAN_POINT ( 'NONE',  ( 0.8499999999999557909, 12.50000000000000000, -6.430097255199264339 ) ) ;
#34224=EDGE_CURVE ( 'NONE', #40462, #32144, #125892, .T. ) ;
#34225=VECTOR ( 'NONE', #2829, 1000.000000000000000 ) ;
#34226=FACE_OUTER_BOUND ( 'NONE', #92690, .T. ) ;
#34227=EDGE_CURVE ( 'NONE', #74400, #70390, #7530, .T. ) ;
#34228=DIRECTION ( 'NONE',  ( -0.000000000000000000, -1.000000000000000000, -0.000000000000000000 ) ) ;
#34229=CONICAL_SURFACE ( 'NONE', #65497, 0.1000000000000000472, 0.003490658503988666988 ) ;
#34230=EDGE_CURVE ( 'NONE', #128842, #128031, #99159, .T. ) ;
#34231=CIRCLE ( 'NONE', #90639, 0.1000000000000002554 ) ;
#34232=ORIENTED_EDGE ( 'NONE', *, *, #86402, .T. ) ;
#34233=CARTESIAN_POINT ( 'NONE',  ( 3.349999999999944578, 2.500000000000000000, -5.802370205355749988 ) ) ;
#34234=VECTOR ( 'NONE', #13346, 1000.000000000000000 ) ;
#34235=EDGE_CURVE ( 'NONE', #116290, #84812, #73665, .T. ) ;
#34236=VERTEX_POINT ( 'NONE', #29760 ) ;
#34237=DIRECTION ( 'NONE',  ( 0.000000000000000000, 1.000000000000000000, 0.000000000000000000 ) ) ;
#34238=VERTEX_POINT ( 'NONE', #17998 ) ;
#34239=CIRCLE ( 'NONE', #19645, 0.06509327318403745899 ) ;
#34240=ADVANCED_FACE ( 'NONE', ( #118138 ), #107682, .T. ) ;
#34241=ORIENTED_EDGE ( 'NONE', *, *, #85591, .T. ) ;
#34243=DIRECTION ( 'NONE',  ( 0.000000000000000000, 0.000000000000000000, 1.000000000000000000 ) ) ;
#34245=DIRECTION ( 'NONE',  ( 0.000000000000000000, 0.000000000000000000, 1.000000000000000000 ) ) ;
#34246=VERTEX_POINT ( 'NONE', #127959 ) ;
#34247=CARTESIAN_POINT ( 'NONE',  ( 9.599999999999917932, 2.500000000000000000, -0.6928203230275541413 ) ) ;
#34248=ORIENTED_EDGE ( 'NONE', *, *, #23892, .T. ) ;
#34249=FACE_OUTER_BOUND ( 'NONE', #46866, .T. ) ;
#34250=DIRECTION ( 'NONE',  ( 0.000000000000000000, 0.000000000000000000, -1.000000000000000000 ) ) ;
#34251=DIRECTION ( 'NONE',  ( 0.000000000000000000, -0.000000000000000000, 1.000000000000000000 ) ) ;
#34252=CARTESIAN_POINT ( 'NONE',  ( -10.85000000000000142, 12.50000000000000000, -5.802370205355746435 ) ) ;
#34253=CIRCLE ( 'NONE', #25823, 0.06509327318403745899 ) ;
#34254=CARTESIAN_POINT ( 'NONE',  ( 5.849999999999932143, 2.500000000000000000, 1.372243186433545370 ) ) ;
#34255=ORIENTED_EDGE ( 'NONE', *, *, #88282, .F. ) ;
#34256=AXIS2_PLACEMENT_3D ( 'NONE', #126670, #87370, #57284 ) ;
#34257=ORIENTED_EDGE ( 'NONE', *, *, #16119, .F. ) ;
#34258=AXIS2_PLACEMENT_3D ( 'NONE', #69542, #87243, #48629 ) ;
#34259=DIRECTION ( 'NONE',  ( -4.274815082592931898E-19, -0.9999939076577903929, -0.003490651415223739937 ) ) ;
#34261=AXIS2_PLACEMENT_3D ( 'NONE', #64524, #96547, #85455 ) ;
#34263=DIRECTION ( 'NONE',  ( -4.274815082592931898E-19, -0.9999939076577903929, -0.003490651415223739937 ) ) ;
#34264=DIRECTION ( 'NONE',  ( -0.000000000000000000, -1.000000000000000000, -0.000000000000000000 ) ) ;
#34266=AXIS2_PLACEMENT_3D ( 'NONE', #89503, #20121, #48293 ) ;
#34268=CONICAL_SURFACE ( 'NONE', #115712, 0.1000000000000002554, 0.003490658503988666988 ) ;
#34269=EDGE_LOOP ( 'NONE', ( #14418, #39641 ) ) ;
#34270=CIRCLE ( 'NONE', #7034, 0.06509327318403741736 ) ;
#34271=CONICAL_SURFACE ( 'NONE', #61460, 0.1000000000000000472, 0.003490658503988666988 ) ;
#34272=DIRECTION ( 'NONE',  ( -0.000000000000000000, -1.000000000000000000, -0.000000000000000000 ) ) ;
#34273=EDGE_CURVE ( 'NONE', #27243, #110807, #78235, .T. ) ;
#34274=CARTESIAN_POINT ( 'NONE',  ( 13.94999999999989804, 2.500000000000000000, 1.718653347947321386 ) ) ;
#34275=DIRECTION ( 'NONE',  ( -0.000000000000000000, 1.000000000000000000, -0.000000000000000000 ) ) ;
#34276=ADVANCED_FACE ( 'NONE', ( #6867 ), #48771, .T. ) ;
#34277=EDGE_LOOP ( 'NONE', ( #3820, #3836, #47819, #69036 ) ) ;
#34278=CIRCLE ( 'NONE', #7046, 0.06509327318403745899 ) ;
#34279=CARTESIAN_POINT ( 'NONE',  ( -7.050000000000016698, 2.500000000000000000, -2.265063509461101798 ) ) ;
#34280=ORIENTED_EDGE ( 'NONE', *, *, #11522, .F. ) ;
#34281=CIRCLE ( 'NONE', #59333, 0.1000000000000002554 ) ;
#34282=CIRCLE ( 'NONE', #32141, 0.1000000000000000056 ) ;
#34283=AXIS2_PLACEMENT_3D ( 'NONE', #17177, #57129, #87225 ) ;
#34284=CARTESIAN_POINT ( 'NONE',  ( 9.549999999999918998, 2.500000000000000000, -6.595190528383302109 ) ) ;
#34285=VECTOR ( 'NONE', #95163, 1000.000000000000000 ) ;
#34287=DIRECTION ( 'NONE',  ( 0.000000000000000000, 0.000000000000000000, -1.000000000000000000 ) ) ;
#34288=DIRECTION ( 'NONE',  ( -0.000000000000000000, 1.000000000000000000, -0.000000000000000000 ) ) ;
#34289=DIRECTION ( 'NONE',  ( 0.000000000000000000, 0.000000000000000000, 1.000000000000000000 ) ) ;
#34290=CIRCLE ( 'NONE', #63525, 0.06509327318403745899 ) ;
#34291=ORIENTED_EDGE ( 'NONE', *, *, #52228, .F. ) ;
#34292=DIRECTION ( 'NONE',  ( -0.000000000000000000, 1.000000000000000000, -0.000000000000000000 ) ) ;
#34293=PLANE ( 'NONE',  #83014 ) ;
#34294=ORIENTED_EDGE ( 'NONE', *, *, #125216, .T. ) ;
#34295=LINE ( 'NONE', #81603, #89178 ) ;
#34296=EDGE_LOOP ( 'NONE', ( #31000, #89529, #88097, #105867 ) ) ;
#34297=ORIENTED_EDGE ( 'NONE', *, *, #127978, .F. ) ;
#34298=DIRECTION ( 'NONE',  ( 0.000000000000000000, 0.000000000000000000, 1.000000000000000000 ) ) ;
#34299=DIRECTION ( 'NONE',  ( 0.000000000000000000, -0.9999939076577903929, 0.003490651415223739937 ) ) ;
#34300=CIRCLE ( 'NONE', #36361, 0.06509327318403745899 ) ;
#34301=DIRECTION ( 'NONE',  ( 0.000000000000000000, 0.000000000000000000, 1.000000000000000000 ) ) ;
#34302=AXIS2_PLACEMENT_3D ( 'NONE', #76501, #86295, #125577 ) ;
#34303=ORIENTED_EDGE ( 'NONE', *, *, #9276, .T. ) ;
#34304=CARTESIAN_POINT ( 'NONE',  ( -7.050000000000013145, 2.500000000000000000, 6.495190528383297135 ) ) ;
#34305=DIRECTION ( 'NONE',  ( -0.000000000000000000, 1.000000000000000000, -0.000000000000000000 ) ) ;
#34306=EDGE_LOOP ( 'NONE', ( #27535, #20791 ) ) ;
#34307=DIRECTION ( 'NONE',  ( -0.000000000000000000, 1.000000000000000000, -0.000000000000000000 ) ) ;
#34308=EDGE_CURVE ( 'NONE', #49236, #59553, #115514, .T. ) ;
#34309=VECTOR ( 'NONE', #85290, 1000.000000000000000 ) ;
#34310=CARTESIAN_POINT ( 'NONE',  ( 3.749999999999976907, 12.50000000000000000, 2.230156782645134950 ) ) ;
#34311=CONICAL_SURFACE ( 'NONE', #111665, 0.1000000000000002554, 0.003490658503988666988 ) ;
#34313=VECTOR ( 'NONE', #111618, 1000.000000000000000 ) ;
#34314=FACE_OUTER_BOUND ( 'NONE', #60316, .T. ) ;
#34315=CARTESIAN_POINT ( 'NONE',  ( 2.500000000000002220, 0.4999999999999993339, 10.00000000000000178 ) ) ;
#34316=CARTESIAN_POINT ( 'NONE',  ( -12.09999999999999432, 2.500000000000000000, 3.637306695894644726 ) ) ;
#34317=PLANE ( 'NONE',  #103665 ) ;
#34318=CARTESIAN_POINT ( 'NONE',  ( -11.64999999999999680, 2.500000000000000000, 6.495190528383297135 ) ) ;
#34319=CONICAL_SURFACE ( 'NONE', #105311, 0.1000000000000002554, 0.003490658503988666988 ) ;
#34320=CONICAL_SURFACE ( 'NONE', #19640, 0.09999999999999982514, 0.003490658503988666988 ) ;
#34321=CIRCLE ( 'NONE', #107462, 0.06509327318403745899 ) ;
#34322=EDGE_LOOP ( 'NONE', ( #94375, #24067 ) ) ;
#34323=VERTEX_POINT ( 'NONE', #37013 ) ;
#34324=EDGE_LOOP ( 'NONE', ( #40903, #62774 ) ) ;
#34325=ORIENTED_EDGE ( 'NONE', *, *, #88728, .F. ) ;
#34326=CARTESIAN_POINT ( 'NONE',  ( -3.750000000000027534, 2.500000000000000000, -1.472243186433550122 ) ) ;
#34327=DIRECTION ( 'NONE',  ( 0.000000000000000000, 0.000000000000000000, -1.000000000000000000 ) ) ;
#34328=ADVANCED_FACE ( 'NONE', ( #67075 ), #46476, .T. ) ;
#34329=CARTESIAN_POINT ( 'NONE',  ( 8.149999999999923972, 12.50000000000000000, 1.818653347947321475 ) ) ;
#34330=ORIENTED_EDGE ( 'NONE', *, *, #55153, .F. ) ;
#34331=FACE_BOUND ( 'NONE', #80032, .T. ) ;
#34333=DIRECTION ( 'NONE',  ( 0.000000000000000000, 0.000000000000000000, -1.000000000000000000 ) ) ;
#34334=DIRECTION ( 'NONE',  ( -0.000000000000000000, 1.000000000000000000, -0.000000000000000000 ) ) ;
#34335=DIRECTION ( 'NONE',  ( -0.000000000000000000, -1.000000000000000000, -0.000000000000000000 ) ) ;
#34336=CARTESIAN_POINT ( 'NONE',  ( 0.6499999999999561684, 2.500000000000000000, -2.511473670974877948 ) ) ;
#34337=LINE ( 'NONE', #14650, #107809 ) ;
#34338=CONICAL_SURFACE ( 'NONE', #11334, 0.1000000000000000472, 0.003490658503988666988 ) ;
#34339=CARTESIAN_POINT ( 'NONE',  ( 14.79999999999989413, 12.50000000000000000, -0.3464101615137782364 ) ) ;
#34340=CARTESIAN_POINT ( 'NONE',  ( 0.8499999999999557909, 12.50000000000000000, -6.495190528383302464 ) ) ;
#34341=DIRECTION ( 'NONE',  ( 0.000000000000000000, 1.000000000000000000, 0.000000000000000000 ) ) ;
#34342=EDGE_CURVE ( 'NONE', #80247, #16543, #96641, .T. ) ;
#34343=CARTESIAN_POINT ( 'NONE',  ( -11.44999999999999751, 2.500000000000000000, 1.818653347947321475 ) ) ;
#34344=CIRCLE ( 'NONE', #86547, 0.09999999999999982514 ) ;
#34345=CARTESIAN_POINT ( 'NONE',  ( 8.949999999999915801, 12.50000000000000000, 6.776507416713035248 ) ) ;
#34346=ORIENTED_EDGE ( 'NONE', *, *, #11627, .T. ) ;
#34347=VERTEX_POINT ( 'NONE', #127331 ) ;
#34348=ORIENTED_EDGE ( 'NONE', *, *, #95197, .F. ) ;
#34349=VERTEX_POINT ( 'NONE', #37663 ) ;
#34351=CARTESIAN_POINT ( 'NONE',  ( 4.599999999999938360, 2.500000000000000000, -0.6928203230275541413 ) ) ;
#34352=ORIENTED_EDGE ( 'NONE', *, *, #19166, .T. ) ;
#34353=ORIENTED_EDGE ( 'NONE', *, *, #14169, .T. ) ;
#34354=AXIS2_PLACEMENT_3D ( 'NONE', #79698, #90144, #120913 ) ;
#34355=DIRECTION ( 'NONE',  ( -0.000000000000000000, -1.000000000000000000, -0.000000000000000000 ) ) ;
#34356=DIRECTION ( 'NONE',  ( 0.000000000000000000, 0.000000000000000000, 1.000000000000000000 ) ) ;
#34357=LINE ( 'NONE', #106299, #76110 ) ;
#34358=CARTESIAN_POINT ( 'NONE',  ( 8.149999999999923972, 2.500000000000000000, -6.148780366869526226 ) ) ;
#34359=ORIENTED_EDGE ( 'NONE', *, *, #35425, .T. ) ;
#34360=CARTESIAN_POINT ( 'NONE',  ( -5.400000000000020783, 2.500000000000000000, 0.5928203230275495006 ) ) ;
#34361=ORIENTED_EDGE ( 'NONE', *, *, #33258, .F. ) ;
#34362=AXIS2_PLACEMENT_3D ( 'NONE', #2867, #53267, #32988 ) ;
#34363=EDGE_CURVE ( 'NONE', #21550, #63883, #128064, .T. ) ;
#34364=ORIENTED_EDGE ( 'NONE', *, *, #106305, .F. ) ;
#34365=CARTESIAN_POINT ( 'NONE',  ( 3.099999999999944134, 2.500000000000000000, 4.676537180435972552 ) ) ;
#34366=ORIENTED_EDGE ( 'NONE', *, *, #124911, .F. ) ;
#34367=LINE ( 'NONE', #76216, #10735 ) ;
#34368=ORIENTED_EDGE ( 'NONE', *, *, #79558, .T. ) ;
#34369=ADVANCED_FACE ( 'NONE', ( #20591 ), #73755, .T. ) ;
#34370=VERTEX_POINT ( 'NONE', #21224 ) ;
#34371=ADVANCED_FACE ( 'NONE', ( #73380 ), #59387, .T. ) ;
#34372=FACE_OUTER_BOUND ( 'NONE', #118359, .T. ) ;
#34373=CARTESIAN_POINT ( 'NONE',  ( 10.59999999999990905, 12.50000000000000000, 4.611443907251934426 ) ) ;
#34374=AXIS2_PLACEMENT_3D ( 'NONE', #89664, #26873, #56955 ) ;
#34375=FACE_OUTER_BOUND ( 'NONE', #119674, .T. ) ;
#34376=CIRCLE ( 'NONE', #82489, 0.06509327318403745899 ) ;
#34377=DIRECTION ( 'NONE',  ( 0.000000000000000000, 0.000000000000000000, 1.000000000000000000 ) ) ;
#34378=ADVANCED_FACE ( 'NONE', ( #80808 ), #13158, .T. ) ;
#34379=ADVANCED_FACE ( 'NONE', ( #53115 ), #100436, .T. ) ;
#34380=CARTESIAN_POINT ( 'NONE',  ( -10.40000000000000213, 12.50000000000000000, -2.276824562219559311E-15 ) ) ;
#34381=AXIS2_PLACEMENT_3D ( 'NONE', #2746, #81952, #32883 ) ;
#34382=EDGE_CURVE ( 'NONE', #100479, #93758, #115614, .T. ) ;
#34383=EDGE_CURVE ( 'NONE', #55744, #113395, #14450, .T. ) ;
#34384=VERTEX_POINT ( 'NONE', #10127 ) ;
#34385=CONICAL_SURFACE ( 'NONE', #71940, 0.09999999999999982514, 0.003490658503988666988 ) ;
#34386=DIRECTION ( 'NONE',  ( -4.274815082592931898E-19, -0.9999939076577903929, -0.003490651415223739937 ) ) ;
#34387=ORIENTED_EDGE ( 'NONE', *, *, #79974, .T. ) ;
#34388=CARTESIAN_POINT ( 'NONE',  ( -3.550000000000028244, 2.500000000000000000, 2.411473670974873862 ) ) ;
#34389=ADVANCED_FACE ( 'NONE', ( #24293 ), #86271, .T. ) ;
#34390=ORIENTED_EDGE ( 'NONE', *, *, #51772, .T. ) ;
#34391=DIRECTION ( 'NONE',  ( 0.000000000000000000, 0.000000000000000000, 1.000000000000000000 ) ) ;
#34392=DIRECTION ( 'NONE',  ( 0.000000000000000000, 0.000000000000000000, 1.000000000000000000 ) ) ;
#34393=CARTESIAN_POINT ( 'NONE',  ( -7.100000000000017408, 2.500000000000000000, -3.537306695894649966 ) ) ;
#34394=PLANE ( 'NONE',  #79405 ) ;
#34395=EDGE_LOOP ( 'NONE', ( #115180, #75181 ) ) ;
#34396=EDGE_CURVE ( 'NONE', #85672, #21815, #17303, .T. ) ;
#34397=FILL_AREA_STYLE_COLOUR ( '', #19369 ) ;
#34398=AXIS2_PLACEMENT_3D ( 'NONE', #111295, #59674, #21658 ) ;
#34399=CONICAL_SURFACE ( 'NONE', #7171, 0.1000000000000002554, 0.003490658503988666988 ) ;
#34400=DIRECTION ( 'NONE',  ( 0.000000000000000000, 1.000000000000000000, 0.000000000000000000 ) ) ;
#34401=ORIENTED_EDGE ( 'NONE', *, *, #120349, .F. ) ;
#34403=AXIS2_PLACEMENT_3D ( 'NONE', #32470, #83485, #1039 ) ;
#34404=AXIS2_PLACEMENT_3D ( 'NONE', #25962, #45610, #113039 ) ;
#34405=ORIENTED_EDGE ( 'NONE', *, *, #53414, .F. ) ;
#34407=DIRECTION ( 'NONE',  ( -0.000000000000000000, 1.000000000000000000, -0.000000000000000000 ) ) ;
#34409=FACE_OUTER_BOUND ( 'NONE', #36314, .T. ) ;
#34410=CIRCLE ( 'NONE', #67827, 0.06509327318403741736 ) ;
#34411=CARTESIAN_POINT ( 'NONE',  ( 7.099999999999927702, 2.500000000000000000, 5.122947341949749323 ) ) ;
#34413=VECTOR ( 'NONE', #25067, 1000.000000000000000 ) ;
#34414=CARTESIAN_POINT ( 'NONE',  ( 11.24999999999994493, 2.500000000000000000, -2.265063509461101798 ) ) ;
#34415=EDGE_LOOP ( 'NONE', ( #50223, #38169 ) ) ;
#34416=AXIS2_PLACEMENT_3D ( 'NONE', #31973, #61438, #3152 ) ;
#34417=LINE ( 'NONE', #63207, #52658 ) ;
#34418=CONICAL_SURFACE ( 'NONE', #61602, 0.1000000000000000472, 0.003490658503988666988 ) ;
#34419=VERTEX_POINT ( 'NONE', #63579 ) ;
#34420=AXIS2_PLACEMENT_3D ( 'NONE', #37763, #76408, #27286 ) ;
#34421=DIRECTION ( 'NONE',  ( -0.000000000000000000, 1.000000000000000000, -0.000000000000000000 ) ) ;
#34422=CARTESIAN_POINT ( 'NONE',  ( -2.100000000000033396, 2.500000000000000000, -0.6928203230275542523 ) ) ;
#34423=DIRECTION ( 'NONE',  ( 0.000000000000000000, 0.000000000000000000, -1.000000000000000000 ) ) ;
#34424=ORIENTED_EDGE ( 'NONE', *, *, #30396, .T. ) ;
#34425=EDGE_CURVE ( 'NONE', #80466, #93509, #48744, .T. ) ;
#34427=CARTESIAN_POINT ( 'NONE',  ( -10.00000000000000533, 2.500000000000000000, 5.122947341949749323 ) ) ;
#34428=AXIS2_PLACEMENT_3D ( 'NONE', #31181, #99907, #118895 ) ;
#34429=ORIENTED_EDGE ( 'NONE', *, *, #48269, .T. ) ;
#34430=DIRECTION ( 'NONE',  ( 0.000000000000000000, 0.000000000000000000, 1.000000000000000000 ) ) ;
#34431=EDGE_CURVE ( 'NONE', #38354, #33550, #82186, .T. ) ;
#34432=VERTEX_POINT ( 'NONE', #34775 ) ;
#34433=EDGE_LOOP ( 'NONE', ( #59984, #54763 ) ) ;
#34434=DIRECTION ( 'NONE',  ( -4.274815082592931898E-19, -0.9999939076577903929, -0.003490651415223739937 ) ) ;
#34435=ORIENTED_EDGE ( 'NONE', *, *, #104993, .F. ) ;
#34436=CARTESIAN_POINT ( 'NONE',  ( 17.17539648375908357, 2.541523116374457825, -5.507477068181845681 ) ) ;
#34437=DIRECTION ( 'NONE',  ( -0.000000000000000000, -1.000000000000000000, -0.000000000000000000 ) ) ;
#34438=AXIS2_PLACEMENT_3D ( 'NONE', #25271, #76333, #74393 ) ;
#34439=CARTESIAN_POINT ( 'NONE',  ( 10.59999999999990905, 12.50000000000000000, 4.676537180435972552 ) ) ;
#34440=AXIS2_PLACEMENT_3D ( 'NONE', #10448, #108647, #110583 ) ;
#34441=ORIENTED_EDGE ( 'NONE', *, *, #79304, .T. ) ;
#34442=LINE ( 'NONE', #14750, #121335 ) ;
#34443=DIRECTION ( 'NONE',  ( -0.000000000000000000, 1.000000000000000000, -0.000000000000000000 ) ) ;
#34444=ORIENTED_EDGE ( 'NONE', *, *, #70093, .T. ) ;
#34445=CARTESIAN_POINT ( 'NONE',  ( 7.699999999999923794, 12.50000000000000000, -0.3464101615137783474 ) ) ;
#34446=FACE_OUTER_BOUND ( 'NONE', #47370, .T. ) ;
#34448=CONICAL_SURFACE ( 'NONE', #105546, 0.09999999999999982514, 0.003490658503988666988 ) ;
#34449=ORIENTED_EDGE ( 'NONE', *, *, #85576, .F. ) ;
#34450=CIRCLE ( 'NONE', #987, 0.06509327318403745899 ) ;
#34451=ORIENTED_EDGE ( 'NONE', *, *, #33628, .T. ) ;
#34452=DIRECTION ( 'NONE',  ( 0.000000000000000000, -0.000000000000000000, 1.000000000000000000 ) ) ;
#34453=DIRECTION ( 'NONE',  ( -0.000000000000000000, 1.000000000000000000, -0.000000000000000000 ) ) ;
#34454=CARTESIAN_POINT ( 'NONE',  ( 2.299999999999948752, 12.50000000000000000, -3.918623584224389056 ) ) ;
#34455=FACE_BOUND ( 'NONE', #62240, .T. ) ;
#34456=VERTEX_POINT ( 'NONE', #44580 ) ;
#34458=DIRECTION ( 'NONE',  ( -0.000000000000000000, -1.000000000000000000, -0.000000000000000000 ) ) ;
#34459=CARTESIAN_POINT ( 'NONE',  ( -11.69999999999999929, 2.500000000000000000, -4.230127018922199333 ) ) ;
#34460=EDGE_CURVE ( 'NONE', #106953, #54196, #29862, .T. ) ;
#34461=DIRECTION ( 'NONE',  ( 0.000000000000000000, 1.000000000000000000, 0.000000000000000000 ) ) ;
#34462=AXIS2_PLACEMENT_3D ( 'NONE', #58916, #117158, #27490 ) ;
#34463=CONICAL_SURFACE ( 'NONE', #122193, 0.1000000000000002554, 0.003490658503988666988 ) ;
#34464=CARTESIAN_POINT ( 'NONE',  ( 5.599999999999934808, 2.500000000000000000, -4.776537180435978414 ) ) ;
#34465=DIRECTION ( 'NONE',  ( 0.000000000000000000, 0.000000000000000000, 1.000000000000000000 ) ) ;
#34466=AXIS2_PLACEMENT_3D ( 'NONE', #92768, #94045, #2417 ) ;
#34467=CARTESIAN_POINT ( 'NONE',  ( 0.3999999999999568345, 2.500000000000000000, -5.022947341949754119 ) ) ;
#34468=AXIS2_PLACEMENT_3D ( 'NONE', #127346, #108956, #10140 ) ;
#34469=ADVANCED_FACE ( 'NONE', ( #50071 ), #96739, .T. ) ;
#34470=DIRECTION ( 'NONE',  ( 0.000000000000000000, 0.000000000000000000, 1.000000000000000000 ) ) ;
#34471=EDGE_LOOP ( 'NONE', ( #91487, #108441, #68860, #18521 ) ) ;
#34472=VERTEX_POINT ( 'NONE', #70333 ) ;
#34474=EDGE_LOOP ( 'NONE', ( #35974, #23621 ) ) ;
#34475=EDGE_LOOP ( 'NONE', ( #51389, #33660, #117029, #109755 ) ) ;
#34476=DIRECTION ( 'NONE',  ( -0.000000000000000000, -1.000000000000000000, -0.000000000000000000 ) ) ;
#34477=EDGE_CURVE ( 'NONE', #94312, #31579, #50686, .T. ) ;
#34478=CARTESIAN_POINT ( 'NONE',  ( 7.299999999999927880, 12.50000000000000000, -4.741630453620015118 ) ) ;
#34479=ORIENTED_EDGE ( 'NONE', *, *, #20566, .T. ) ;
#34480=FACE_BOUND ( 'NONE', #3661, .T. ) ;
#34481=EDGE_CURVE ( 'NONE', #79643, #37274, #128157, .T. ) ;
#34482=DIRECTION ( 'NONE',  ( 0.000000000000000000, 0.000000000000000000, 1.000000000000000000 ) ) ;
#34483=AXIS2_PLACEMENT_3D ( 'NONE', #26810, #8436, #55621 ) ;
#34484=EDGE_CURVE ( 'NONE', #107557, #84136, #71716, .T. ) ;
#34485=FACE_OUTER_BOUND ( 'NONE', #115085, .T. ) ;
#34486=AXIS2_PLACEMENT_3D ( 'NONE', #83500, #23258, #123398 ) ;
#34487=CONICAL_SURFACE ( 'NONE', #19803, 0.1000000000000002554, 0.003490658503988666988 ) ;
#34488=EDGE_LOOP ( 'NONE', ( #3482, #37452, #116047, #94557 ) ) ;
#34489=AXIS2_PLACEMENT_3D ( 'NONE', #46892, #67807, #106443 ) ;
#34490=DIRECTION ( 'NONE',  ( 0.000000000000000000, 0.000000000000000000, 1.000000000000000000 ) ) ;
#34491=PLANE ( 'NONE',  #128545 ) ;
#34492=EDGE_CURVE ( 'NONE', #81402, #109700, #11058, .T. ) ;
#34493=CARTESIAN_POINT ( 'NONE',  ( -2.950000000000033484, 2.500000000000000000, -6.495190528383302464 ) ) ;
#34494=ORIENTED_EDGE ( 'NONE', *, *, #99087, .F. ) ;
#34495=DIRECTION ( 'NONE',  ( 0.000000000000000000, 1.000000000000000000, 0.000000000000000000 ) ) ;
#34496=EDGE_LOOP ( 'NONE', ( #60550, #95055, #12230, #88190 ) ) ;
#34497=AXIS2_PLACEMENT_3D ( 'NONE', #3257, #121091, #43199 ) ;
#34498=CIRCLE ( 'NONE', #59556, 0.1000000000000002554 ) ;
#34499=ORIENTED_EDGE ( 'NONE', *, *, #54173, .F. ) ;
#34500=ORIENTED_EDGE ( 'NONE', *, *, #82769, .T. ) ;
#34501=DIRECTION ( 'NONE',  ( 0.000000000000000000, 0.000000000000000000, 1.000000000000000000 ) ) ;
#34502=AXIS2_PLACEMENT_3D ( 'NONE', #122312, #32659, #13617 ) ;
#34503=FACE_OUTER_BOUND ( 'NONE', #73093, .T. ) ;
#34504=LINE ( 'NONE', #114326, #4905 ) ;
#34505=VERTEX_POINT ( 'NONE', #96890 ) ;
#34506=CARTESIAN_POINT ( 'NONE',  ( 5.399999999999936406, 2.500000000000000000, -3.737306695894649700 ) ) ;
#34507=CONICAL_SURFACE ( 'NONE', #74198, 0.1000000000000002554, 0.003490658503988666988 ) ;
#34508=CIRCLE ( 'NONE', #51228, 0.09999999999999982514 ) ;
#34509=CARTESIAN_POINT ( 'NONE',  ( -8.550000000000013145, 12.50000000000000000, -1.818653347947326138 ) ) ;
#34510=DIRECTION ( 'NONE',  ( 0.000000000000000000, 1.000000000000000000, 0.000000000000000000 ) ) ;
#34512=CARTESIAN_POINT ( 'NONE',  ( -5.850000000000019185, 12.50000000000000000, 2.165063509461097713 ) ) ;
#34513=VECTOR ( 'NONE', #126479, 1000.000000000000000 ) ;
#34514=VERTEX_POINT ( 'NONE', #6537 ) ;
#34515=CARTESIAN_POINT ( 'NONE',  ( -12.09999999999999609, 2.500000000000000000, -3.737306695894647035 ) ) ;
#34516=ORIENTED_EDGE ( 'NONE', *, *, #97301, .F. ) ;
#34517=CARTESIAN_POINT ( 'NONE',  ( 1.249999999999952038, 2.500000000000000000, -1.472243186433550122 ) ) ;
#34518=ORIENTED_EDGE ( 'NONE', *, *, #3044, .F. ) ;
#34519=EDGE_LOOP ( 'NONE', ( #50927, #62622, #113791, #13421 ) ) ;
#34520=DIRECTION ( 'NONE',  ( -0.000000000000000000, -1.000000000000000000, -0.000000000000000000 ) ) ;
#34521=DIRECTION ( 'NONE',  ( -0.000000000000000000, -1.000000000000000000, -0.000000000000000000 ) ) ;
#34522=DIRECTION ( 'NONE',  ( 0.000000000000000000, 0.000000000000000000, 1.000000000000000000 ) ) ;
#34523=DIRECTION ( 'NONE',  ( 0.000000000000000000, 0.000000000000000000, 1.000000000000000000 ) ) ;
#34525=VECTOR ( 'NONE', #78103, 1000.000000000000000 ) ;
#34526=EDGE_LOOP ( 'NONE', ( #122032, #48125, #106749, #80097 ) ) ;
#34528=EDGE_CURVE ( 'NONE', #56626, #106131, #16374, .T. ) ;
#34529=FACE_OUTER_BOUND ( 'NONE', #49078, .T. ) ;
#34530=CARTESIAN_POINT ( 'NONE',  ( 1.849999999999950129, 12.50000000000000000, -6.776507416713040577 ) ) ;
#34531=CARTESIAN_POINT ( 'NONE',  ( 3.949999999999940670, 2.500000000000000000, 1.818653347947321475 ) ) ;
#34532=ADVANCED_FACE ( 'NONE', ( #27486 ), #46497, .T. ) ;
#34533=EDGE_LOOP ( 'NONE', ( #12915, #77634 ) ) ;
#34534=ORIENTED_EDGE ( 'NONE', *, *, #61817, .T. ) ;
#34535=ADVANCED_FACE ( 'NONE', ( #127646 ), #35410, .T. ) ;
#34536=LINE ( 'NONE', #64612, #12290 ) ;
#34537=ADVANCED_FACE ( 'NONE', ( #125069 ), #52843, .T. ) ;
#34538=CIRCLE ( 'NONE', #122357, 0.06509327318403741736 ) ;
#34539=EDGE_CURVE ( 'NONE', #61976, #20692, #44521, .T. ) ;
#34540=ORIENTED_EDGE ( 'NONE', *, *, #36591, .T. ) ;
#34541=CARTESIAN_POINT ( 'NONE',  ( -12.89999999999999147, 12.50000000000000000, -4.957854068765714217 ) ) ;
#34542=AXIS2_PLACEMENT_3D ( 'NONE', #90790, #121525, #52796 ) ;
#34543=CARTESIAN_POINT ( 'NONE',  ( 6.699999999999930012, 12.50000000000000000, 4.330127018922196314 ) ) ;
#34544=ORIENTED_EDGE ( 'NONE', *, *, #73933, .F. ) ;
#34545=FACE_OUTER_BOUND ( 'NONE', #16462, .T. ) ;
#34546=EDGE_CURVE ( 'NONE', #110045, #101913, #121888, .T. ) ;
#34547=CARTESIAN_POINT ( 'NONE',  ( -8.350000000000010303, 2.500000000000000000, 6.495190528383297135 ) ) ;
#34548=CARTESIAN_POINT ( 'NONE',  ( -12.49999999999999467, 12.50000000000000000, 0.6928203230275535862 ) ) ;
#34549=DIRECTION ( 'NONE',  ( -0.000000000000000000, 1.000000000000000000, -0.000000000000000000 ) ) ;
#34550=ORIENTED_EDGE ( 'NONE', *, *, #94189, .T. ) ;
#34551=EDGE_CURVE ( 'NONE', #18774, #127039, #50954, .T. ) ;
#34552=AXIS2_PLACEMENT_3D ( 'NONE', #28963, #99628, #98977 ) ;
#34553=FACE_OUTER_BOUND ( 'NONE', #96154, .T. ) ;
#34554=EDGE_CURVE ( 'NONE', #31546, #45780, #2646, .T. ) ;
#34555=DIRECTION ( 'NONE',  ( 0.000000000000000000, 1.000000000000000000, 0.000000000000000000 ) ) ;
#34556=AXIS2_PLACEMENT_3D ( 'NONE', #35913, #75828, #115756 ) ;
#34557=VERTEX_POINT ( 'NONE', #77261 ) ;
#34558=ORIENTED_EDGE ( 'NONE', *, *, #31268, .T. ) ;
#34559=DIRECTION ( 'NONE',  ( -0.000000000000000000, -1.000000000000000000, -0.000000000000000000 ) ) ;
#34560=DIRECTION ( 'NONE',  ( -0.000000000000000000, -1.000000000000000000, -0.000000000000000000 ) ) ;
#34561=CARTESIAN_POINT ( 'NONE',  ( -11.69999999999999929, 2.500000000000000000, -0.09999999999999827083 ) ) ;
#34562=DIRECTION ( 'NONE',  ( -0.000000000000000000, 1.000000000000000000, -0.000000000000000000 ) ) ;
#34563=LINE ( 'NONE', #74466, #123809 ) ;
#34564=VECTOR ( 'NONE', #45567, 1000.000000000000000 ) ;
#34565=PLANE ( 'NONE',  #115757 ) ;
#34566=DIRECTION ( 'NONE',  ( 0.000000000000000000, 0.000000000000000000, 1.000000000000000000 ) ) ;
#34568=DIRECTION ( 'NONE',  ( 0.000000000000000000, 0.000000000000000000, 1.000000000000000000 ) ) ;
#34569=ADVANCED_FACE ( 'NONE', ( #85135 ), #123929, .T. ) ;
#34570=DIRECTION ( 'NONE',  ( 0.000000000000000000, 0.000000000000000000, 1.000000000000000000 ) ) ;
#34571=ORIENTED_EDGE ( 'NONE', *, *, #11569, .F. ) ;
#34572=ORIENTED_EDGE ( 'NONE', *, *, #109163, .T. ) ;
#34573=EDGE_LOOP ( 'NONE', ( #72766, #70506, #97060, #26551 ) ) ;
#34574=ORIENTED_EDGE ( 'NONE', *, *, #77661, .F. ) ;
#34575=CARTESIAN_POINT ( 'NONE',  ( 8.749999999999923617, 12.50000000000000000, 1.537336459617582918 ) ) ;
#34576=AXIS2_PLACEMENT_3D ( 'NONE', #119832, #31464, #70735 ) ;
#34577=CARTESIAN_POINT ( 'NONE',  ( 8.749999999999920064, 12.50000000000000000, 5.802370205355744659 ) ) ;
#34578=LINE ( 'NONE', #78198, #31305 ) ;
#34580=CARTESIAN_POINT ( 'NONE',  ( 9.999999999999948486, 12.50000000000000000, 4.330127018922196314 ) ) ;
#34581=VECTOR ( 'NONE', #113756, 1000.000000000000000 ) ;
#34582=AXIS2_PLACEMENT_3D ( 'NONE', #116154, #26508, #114865 ) ;
#34583=CARTESIAN_POINT ( 'NONE',  ( -0.4000000000000404898, 2.500000000000000000, 5.122947341949749323 ) ) ;
#34584=CARTESIAN_POINT ( 'NONE',  ( -5.400000000000020783, 2.500000000000000000, 0.6928203230275494784 ) ) ;
#34585=ORIENTED_EDGE ( 'NONE', *, *, #95097, .F. ) ;
#34586=AXIS2_PLACEMENT_3D ( 'NONE', #89078, #119818, #67467 ) ;
#34587=PLANE ( 'NONE',  #49519 ) ;
#34588=LINE ( 'NONE', #88658, #56289 ) ;
#34589=ORIENTED_EDGE ( 'NONE', *, *, #13458, .F. ) ;
#34591=EDGE_CURVE ( 'NONE', #114219, #22468, #104758, .T. ) ;
#34592=CIRCLE ( 'NONE', #22066, 0.1000000000000002554 ) ;
#34593=VECTOR ( 'NONE', #57056, 1000.000000000000000 ) ;
#34594=VERTEX_POINT ( 'NONE', #5281 ) ;
#34595=VERTEX_POINT ( 'NONE', #47809 ) ;
#34596=EDGE_LOOP ( 'NONE', ( #9918, #100791, #42568, #47203 ) ) ;
#34597=DIRECTION ( 'NONE',  ( -0.000000000000000000, 1.000000000000000000, -0.000000000000000000 ) ) ;
#34598=VECTOR ( 'NONE', #102503, 1000.000000000000000 ) ;
#34599=CARTESIAN_POINT ( 'NONE',  ( -7.500000000000015099, 2.500000000000000000, -5.122947341949753763 ) ) ;
#34600=DIRECTION ( 'NONE',  ( 0.000000000000000000, 1.000000000000000000, 0.000000000000000000 ) ) ;
#34601=CONICAL_SURFACE ( 'NONE', #111952, 0.1000000000000000472, 0.003490658503988666988 ) ;
#34602=DIRECTION ( 'NONE',  ( 0.000000000000000000, 0.000000000000000000, 1.000000000000000000 ) ) ;
#34604=ORIENTED_EDGE ( 'NONE', *, *, #1535, .T. ) ;
#34605=CIRCLE ( 'NONE', #13726, 0.06509327318403745899 ) ;
#34606=DIRECTION ( 'NONE',  ( 0.000000000000000000, 0.000000000000000000, 1.000000000000000000 ) ) ;
#34607=VECTOR ( 'NONE', #23601, 1000.000000000000000 ) ;
#34608=EDGE_LOOP ( 'NONE', ( #93033, #126995 ) ) ;
#34610=DIRECTION ( 'NONE',  ( 0.000000000000000000, 0.000000000000000000, 1.000000000000000000 ) ) ;
#34611=DIRECTION ( 'NONE',  ( 0.000000000000000000, 1.000000000000000000, 0.000000000000000000 ) ) ;
#34612=FACE_OUTER_BOUND ( 'NONE', #66922, .T. ) ;
#34613=EDGE_LOOP ( 'NONE', ( #120287, #95862, #16263, #58295 ) ) ;
#34614=VERTEX_POINT ( 'NONE', #85775 ) ;
#34615=ORIENTED_EDGE ( 'NONE', *, *, #58700, .T. ) ;
#34616=DIRECTION ( 'NONE',  ( -0.000000000000000000, -1.000000000000000000, -0.000000000000000000 ) ) ;
#34617=CARTESIAN_POINT ( 'NONE',  ( 8.749999999999957367, 2.500000000000000000, 2.165063509461097713 ) ) ;
#34618=CARTESIAN_POINT ( 'NONE',  ( 4.149999999999941735, 12.50000000000000000, -5.802370205355749988 ) ) ;
#34619=FACE_BOUND ( 'NONE', #43257, .T. ) ;
#34620=CARTESIAN_POINT ( 'NONE',  ( 1.649999999999950617, 12.50000000000000000, -2.165063509461101710 ) ) ;
#34621=VECTOR ( 'NONE', #50405, 1000.000000000000000 ) ;
#34622=DIRECTION ( 'NONE',  ( 0.000000000000000000, 0.000000000000000000, -1.000000000000000000 ) ) ;
#34623=FACE_OUTER_BOUND ( 'NONE', #45983, .T. ) ;
#34624=DIRECTION ( 'NONE',  ( 0.000000000000000000, 0.000000000000000000, -1.000000000000000000 ) ) ;
#34625=VECTOR ( 'NONE', #52498, 1000.000000000000000 ) ;
#34626=LINE ( 'NONE', #95460, #119834 ) ;
#34627=DIRECTION ( 'NONE',  ( 0.000000000000000000, 0.000000000000000000, -1.000000000000000000 ) ) ;
#34628=ORIENTED_EDGE ( 'NONE', *, *, #68294, .T. ) ;
#34629=CIRCLE ( 'NONE', #15814, 0.1000000000000000472 ) ;
#34630=AXIS2_PLACEMENT_3D ( 'NONE', #34467, #124110, #114294 ) ;
#34631=EDGE_CURVE ( 'NONE', #92907, #81402, #37974, .T. ) ;
#34632=CARTESIAN_POINT ( 'NONE',  ( 13.09999999999990195, 12.50000000000000000, -4.048810130592463530 ) ) ;
#34633=EDGE_LOOP ( 'NONE', ( #75603, #100190, #66654, #16193 ) ) ;
#34635=VERTEX_POINT ( 'NONE', #55038 ) ;
#34636=ORIENTED_EDGE ( 'NONE', *, *, #33478, .F. ) ;
#34637=ADVANCED_FACE ( 'NONE', ( #94973 ), #45229, .T. ) ;
#34638=CARTESIAN_POINT ( 'NONE',  ( 11.04999999999990834, 12.50000000000000000, 1.818653347947321475 ) ) ;
#34639=FACE_BOUND ( 'NONE', #77585, .T. ) ;
#34640=ADVANCED_FACE ( 'NONE', ( #5912 ), #69558, .T. ) ;
#34641=DIRECTION ( 'NONE',  ( 0.000000000000000000, -0.9999939076577903929, 0.003490651415223739937 ) ) ;
#34642=AXIS2_PLACEMENT_3D ( 'NONE', #98171, #120407, #30107 ) ;
#34643=AXIS2_PLACEMENT_3D ( 'NONE', #24013, #113026, #46221 ) ;
#34644=EDGE_CURVE ( 'NONE', #72427, #80727, #29456, .T. ) ;
#34645=ADVANCED_FACE ( 'NONE', ( #51040 ), #65443, .T. ) ;
#34646=ORIENTED_EDGE ( 'NONE', *, *, #85580, .T. ) ;
#34647=FACE_OUTER_BOUND ( 'NONE', #4325, .T. ) ;
#34648=EDGE_CURVE ( 'NONE', #32199, #124072, #81138, .T. ) ;
#34649=EDGE_CURVE ( 'NONE', #127662, #129312, #46573, .T. ) ;
#34650=DIRECTION ( 'NONE',  ( 0.000000000000000000, 0.000000000000000000, 1.000000000000000000 ) ) ;
#34651=EDGE_CURVE ( 'NONE', #111888, #31897, #48440, .T. ) ;
#34652=ORIENTED_EDGE ( 'NONE', *, *, #117690, .F. ) ;
#34653=CARTESIAN_POINT ( 'NONE',  ( -2.499999999999996003, 12.50000000000000000, -4.330127018922201643 ) ) ;
#34654=DIRECTION ( 'NONE',  ( 0.000000000000000000, 0.000000000000000000, -1.000000000000000000 ) ) ;
#34655=AXIS2_PLACEMENT_3D ( 'NONE', #77435, #125875, #57150 ) ;
#34656=CIRCLE ( 'NONE', #13685, 0.06509327318403745899 ) ;
#34657=ORIENTED_EDGE ( 'NONE', *, *, #41151, .T. ) ;
#34658=DIRECTION ( 'NONE',  ( -0.000000000000000000, -1.000000000000000000, -0.000000000000000000 ) ) ;
#34659=CARTESIAN_POINT ( 'NONE',  ( -11.84999999999999609, 12.50000000000000000, 6.776507416713035248 ) ) ;
#34660=EDGE_CURVE ( 'NONE', #28229, #6619, #9007, .T. ) ;
#34661=VERTEX_POINT ( 'NONE', #39305 ) ;
#34662=CARTESIAN_POINT ( 'NONE',  ( -8.550000000000009592, 2.500000000000000000, 6.841600689897072485 ) ) ;
#34663=DIRECTION ( 'NONE',  ( -0.000000000000000000, -1.000000000000000000, -0.000000000000000000 ) ) ;
#34664=DIRECTION ( 'NONE',  ( 0.000000000000000000, 0.000000000000000000, 1.000000000000000000 ) ) ;
#34665=EDGE_LOOP ( 'NONE', ( #126513, #80238 ) ) ;
#34666=EDGE_LOOP ( 'NONE', ( #32063, #51547, #33114, #94626 ) ) ;
#34667=LINE ( 'NONE', #123644, #45174 ) ;
#34668=CIRCLE ( 'NONE', #18390, 0.06509327318403745899 ) ;
#34669=ORIENTED_EDGE ( 'NONE', *, *, #124964, .F. ) ;
#34670=DIRECTION ( 'NONE',  ( 0.000000000000000000, 0.000000000000000000, -1.000000000000000000 ) ) ;
#34671=DIRECTION ( 'NONE',  ( -0.000000000000000000, -1.000000000000000000, -0.000000000000000000 ) ) ;
#34672=AXIS2_PLACEMENT_3D ( 'NONE', #120616, #2118, #30971 ) ;
#34674=CIRCLE ( 'NONE', #124545, 0.06509327318403745899 ) ;
#34675=DIRECTION ( 'NONE',  ( 0.000000000000000000, 1.000000000000000000, 0.000000000000000000 ) ) ;
#34677=CARTESIAN_POINT ( 'NONE',  ( -5.800000000000022027, 12.50000000000000000, -4.265033745738164406 ) ) ;
#34678=CARTESIAN_POINT ( 'NONE',  ( -4.600000000000025402, 12.50000000000000000, -2.385244779468109755E-15 ) ) ;
#34679=FACE_OUTER_BOUND ( 'NONE', #87599, .T. ) ;
#34680=EDGE_LOOP ( 'NONE', ( #57204, #39863 ) ) ;
#34681=VERTEX_POINT ( 'NONE', #621 ) ;
#34682=CARTESIAN_POINT ( 'NONE',  ( -6.900000000000019007, 12.50000000000000000, 0.4115034346978109769 ) ) ;
#34684=DIRECTION ( 'NONE',  ( 0.000000000000000000, 0.000000000000000000, 1.000000000000000000 ) ) ;
#34685=AXIS2_PLACEMENT_3D ( 'NONE', #48098, #89305, #61139 ) ;
#34686=ORIENTED_EDGE ( 'NONE', *, *, #103965, .F. ) ;
#34687=VERTEX_POINT ( 'NONE', #40589 ) ;
#34688=ORIENTED_EDGE ( 'NONE', *, *, #42840, .T. ) ;
#34689=EDGE_CURVE ( 'NONE', #66521, #74881, #21544, .T. ) ;
#34690=DIRECTION ( 'NONE',  ( -0.000000000000000000, 1.000000000000000000, -0.000000000000000000 ) ) ;
#34691=ADVANCED_FACE ( 'NONE', ( #30115 ), #23591, .T. ) ;
#34692=CIRCLE ( 'NONE', #7466, 0.06509327318403745899 ) ;
#34693=DIRECTION ( 'NONE',  ( -0.000000000000000000, 1.000000000000000000, -0.000000000000000000 ) ) ;
#34694=AXIS2_PLACEMENT_3D ( 'NONE', #47856, #10482, #70063 ) ;
#34696=ADVANCED_FACE ( 'NONE', ( #108001 ), #89661, .T. ) ;
#34698=CARTESIAN_POINT ( 'NONE',  ( 11.64999999999990798, 2.500000000000000000, -1.472243186433550122 ) ) ;
#34699=DIRECTION ( 'NONE',  ( 0.000000000000000000, 0.000000000000000000, -1.000000000000000000 ) ) ;
#34700=FACE_OUTER_BOUND ( 'NONE', #1452, .T. ) ;
#34701=CONICAL_SURFACE ( 'NONE', #61883, 0.1000000000000002554, 0.003490658503988666988 ) ;
#34702=CARTESIAN_POINT ( 'NONE',  ( -8.350000000000008527, 12.50000000000000000, 5.802370205355744659 ) ) ;
#34703=CARTESIAN_POINT ( 'NONE',  ( -0.6500000000000394351, 12.50000000000000000, 6.906693963081109722 ) ) ;
#34704=EDGE_CURVE ( 'NONE', #70719, #14663, #65541, .T. ) ;
#34705=DIRECTION ( 'NONE',  ( 0.000000000000000000, 1.000000000000000000, 0.000000000000000000 ) ) ;
#34706=ADVANCED_FACE ( 'NONE', ( #41225 ), #70658, .T. ) ;
#34707=EDGE_CURVE ( 'NONE', #10760, #47322, #84327, .T. ) ;
#34708=VERTEX_POINT ( 'NONE', #18329 ) ;
#34709=EDGE_CURVE ( 'NONE', #37316, #96170, #58275, .T. ) ;
#34710=DIRECTION ( 'NONE',  ( -0.000000000000000000, -1.000000000000000000, -0.000000000000000000 ) ) ;
#34711=VERTEX_POINT ( 'NONE', #39928 ) ;
#34712=ORIENTED_EDGE ( 'NONE', *, *, #112530, .T. ) ;
#34713=CARTESIAN_POINT ( 'NONE',  ( 1.049999999999954525, 2.500000000000000000, -2.511473670974877948 ) ) ;
#34714=CARTESIAN_POINT ( 'NONE',  ( 10.59999999999990905, 12.50000000000000000, -3.918623584224389056 ) ) ;
#34715=AXIS2_PLACEMENT_3D ( 'NONE', #43839, #61536, #92930 ) ;
#34716=FACE_OUTER_BOUND ( 'NONE', #32504, .T. ) ;
#34717=ADVANCED_FACE ( 'NONE', ( #118463 ), #9108, .T. ) ;
#34718=DIRECTION ( 'NONE',  ( 0.000000000000000000, 0.000000000000000000, 1.000000000000000000 ) ) ;
#34719=CARTESIAN_POINT ( 'NONE',  ( 0.3999999999999628852, 2.500000000000000000, -0.6928203230275520319 ) ) ;
#34720=DIRECTION ( 'NONE',  ( -0.000000000000000000, -1.000000000000000000, -0.000000000000000000 ) ) ;
#34721=DIRECTION ( 'NONE',  ( 0.000000000000000000, 1.000000000000000000, 0.000000000000000000 ) ) ;
#34722=ORIENTED_EDGE ( 'NONE', *, *, #23697, .F. ) ;
#34723=CARTESIAN_POINT ( 'NONE',  ( -7.500000000000001776, -2.500000000000000000, 1.734723475976807094E-15 ) ) ;
#34724=AXIS2_PLACEMENT_3D ( 'NONE', #88387, #128358, #96277 ) ;
#34725=AXIS2_PLACEMENT_3D ( 'NONE', #2236, #93858, #42186 ) ;
#34726=VECTOR ( 'NONE', #129303, 1000.000000000000000 ) ;
#34727=CARTESIAN_POINT ( 'NONE',  ( 4.549999999999935874, 2.500000000000000000, 6.395190528383296602 ) ) ;
#34728=EDGE_LOOP ( 'NONE', ( #110697, #115894 ) ) ;
#34729=VERTEX_POINT ( 'NONE', #108646 ) ;
#34730=AXIS2_PLACEMENT_3D ( 'NONE', #13013, #91604, #102073 ) ;
#34731=ORIENTED_EDGE ( 'NONE', *, *, #22390, .F. ) ;
#34732=EDGE_CURVE ( 'NONE', #52697, #108629, #89021, .T. ) ;
#34733=ORIENTED_EDGE ( 'NONE', *, *, #110712, .F. ) ;
#34734=CARTESIAN_POINT ( 'NONE',  ( 0.5999999999999547917, 12.50000000000000000, 3.983716857408420076 ) ) ;
#34735=DIRECTION ( 'NONE',  ( 0.000000000000000000, 1.000000000000000000, 0.000000000000000000 ) ) ;
#34736=DIRECTION ( 'NONE',  ( -0.000000000000000000, 1.000000000000000000, -0.000000000000000000 ) ) ;
#34737=FACE_OUTER_BOUND ( 'NONE', #79348, .T. ) ;
#34738=AXIS2_PLACEMENT_3D ( 'NONE', #7117, #126267, #105980 ) ;
#34739=AXIS2_PLACEMENT_3D ( 'NONE', #51877, #32251, #73427 ) ;
#34740=DIRECTION ( 'NONE',  ( 0.000000000000000000, 0.000000000000000000, 1.000000000000000000 ) ) ;
#34741=VERTEX_POINT ( 'NONE', #109292 ) ;
#34742=DIRECTION ( 'NONE',  ( -0.000000000000000000, -1.000000000000000000, -0.000000000000000000 ) ) ;
#34743=FACE_OUTER_BOUND ( 'NONE', #63152, .T. ) ;
#34744=CARTESIAN_POINT ( 'NONE',  ( 1.249999999999950262, 12.50000000000000000, 7.188010851410848723 ) ) ;
#34745=ORIENTED_EDGE ( 'NONE', *, *, #114540, .F. ) ;
#34748=EDGE_LOOP ( 'NONE', ( #77572, #84686 ) ) ;
#34749=CARTESIAN_POINT ( 'NONE',  ( 10.19999999999991047, 12.50000000000000000, -3.983716857408426293 ) ) ;
#34750=FACE_OUTER_BOUND ( 'NONE', #109161, .T. ) ;
#34751=DIRECTION ( 'NONE',  ( 0.000000000000000000, -0.9999939076577903929, 0.003490651415223739937 ) ) ;
#34752=ORIENTED_EDGE ( 'NONE', *, *, #103491, .F. ) ;
#34753=DIRECTION ( 'NONE',  ( -0.000000000000000000, 1.000000000000000000, -0.000000000000000000 ) ) ;
#34754=DIRECTION ( 'NONE',  ( 0.000000000000000000, 0.000000000000000000, 1.000000000000000000 ) ) ;
#34755=ADVANCED_FACE ( 'NONE', ( #111207 ), #27892, .T. ) ;
#34756=CARTESIAN_POINT ( 'NONE',  ( -5.850000000000019185, 12.50000000000000000, 6.430097255199259010 ) ) ;
#34757=DIRECTION ( 'NONE',  ( -4.274815082592931898E-19, -0.9999939076577903929, -0.003490651415223739937 ) ) ;
#34758=LINE ( 'NONE', #74022, #5928 ) ;
#34759=ORIENTED_EDGE ( 'NONE', *, *, #23495, .T. ) ;
#34760=AXIS2_PLACEMENT_3D ( 'NONE', #124491, #104195, #14508 ) ;
#34761=DIRECTION ( 'NONE',  ( 0.000000000000000000, -0.9999939076577903929, 0.003490651415223739937 ) ) ;
#34762=VECTOR ( 'NONE', #68187, 1000.000000000000000 ) ;
#34763=ORIENTED_EDGE ( 'NONE', *, *, #48450, .F. ) ;
#34764=ORIENTED_EDGE ( 'NONE', *, *, #52542, .T. ) ;
#34765=DIRECTION ( 'NONE',  ( -0.000000000000000000, -1.000000000000000000, -0.000000000000000000 ) ) ;
#34766=CARTESIAN_POINT ( 'NONE',  ( 12.69999999999990337, 12.50000000000000000, 3.983716857408420076 ) ) ;
#34767=CARTESIAN_POINT ( 'NONE',  ( 6.699999999999928235, 12.50000000000000000, -2.276824562219559311E-15 ) ) ;
#34768=FACE_OUTER_BOUND ( 'NONE', #78763, .T. ) ;
#34769=AXIS2_PLACEMENT_3D ( 'NONE', #127506, #26090, #97388 ) ;
#34770=DIRECTION ( 'NONE',  ( 0.000000000000000000, 1.000000000000000000, 0.000000000000000000 ) ) ;
#34771=ORIENTED_EDGE ( 'NONE', *, *, #85632, .F. ) ;
#34772=VERTEX_POINT ( 'NONE', #123612 ) ;
#34773=DIRECTION ( 'NONE',  ( 0.000000000000000000, 1.000000000000000000, 0.000000000000000000 ) ) ;
#34774=FACE_OUTER_BOUND ( 'NONE', #84918, .T. ) ;
#34775=CARTESIAN_POINT ( 'NONE',  ( 0.4499999999999569344, 12.50000000000000000, 2.099970236277060032 ) ) ;
#34776=DIRECTION ( 'NONE',  ( 0.000000000000000000, 0.000000000000000000, 1.000000000000000000 ) ) ;
#34777=VERTEX_POINT ( 'NONE', #23488 ) ;
#34778=CIRCLE ( 'NONE', #101671, 0.09999999999999982514 ) ;
#34779=LINE ( 'NONE', #66145, #7146 ) ;
#34780=AXIS2_PLACEMENT_3D ( 'NONE', #123218, #114666, #25006 ) ;
#34782=CARTESIAN_POINT ( 'NONE',  ( 8.749999999999953815, 12.50000000000000000, -2.165063509461101710 ) ) ;
#34783=VERTEX_POINT ( 'NONE', #14301 ) ;
#34784=CARTESIAN_POINT ( 'NONE',  ( 4.349999999999940137, 12.50000000000000000, -6.776507416713040577 ) ) ;
#34785=ORIENTED_EDGE ( 'NONE', *, *, #98631, .F. ) ;
#34786=FACE_BOUND ( 'NONE', #114515, .T. ) ;
#34788=DIRECTION ( 'NONE',  ( 0.000000000000000000, 0.000000000000000000, -1.000000000000000000 ) ) ;
#34789=ORIENTED_EDGE ( 'NONE', *, *, #52356, .F. ) ;
#34790=CARTESIAN_POINT ( 'NONE',  ( 3.099999999999943245, 12.50000000000000000, 3.983716857408420076 ) ) ;
#34791=FACE_OUTER_BOUND ( 'NONE', #82993, .T. ) ;
#34792=ADVANCED_FACE ( 'NONE', ( #53608 ), #13001, .T. ) ;
#34795=ORIENTED_EDGE ( 'NONE', *, *, #82505, .F. ) ;
#34796=ADVANCED_FACE ( 'NONE', ( #32699 ), #94795, .T. ) ;
#34797=ADVANCED_FACE ( 'NONE', ( #103356 ), #113579, .T. ) ;
#34799=AXIS2_PLACEMENT_3D ( 'NONE', #28047, #98063, #10335 ) ;
#34801=CARTESIAN_POINT ( 'NONE',  ( 3.149999999999942624, 2.500000000000000000, 6.841600689897072485 ) ) ;
#34802=AXIS2_PLACEMENT_3D ( 'NONE', #9478, #47471, #87376 ) ;
#34803=FACE_OUTER_BOUND ( 'NONE', #122048, .T. ) ;
#34804=DIRECTION ( 'NONE',  ( 0.000000000000000000, 0.000000000000000000, 1.000000000000000000 ) ) ;
#34805=CARTESIAN_POINT ( 'NONE',  ( -10.65000000000000391, 12.50000000000000000, -6.906693963081112386 ) ) ;
#34806=AXIS2_PLACEMENT_3D ( 'NONE', #36601, #86960, #46380 ) ;
#34807=PLANE ( 'NONE',  #79870 ) ;
#34808=EDGE_CURVE ( 'NONE', #30916, #25579, #698, .T. ) ;
#34809=AXIS2_PLACEMENT_3D ( 'NONE', #96258, #84525, #124455 ) ;
#34810=AXIS2_PLACEMENT_3D ( 'NONE', #36883, #108818, #39480 ) ;
#34811=EDGE_CURVE ( 'NONE', #62130, #14341, #80129, .T. ) ;
#34812=EDGE_CURVE ( 'NONE', #4541, #17715, #91592, .T. ) ;
#34813=ORIENTED_EDGE ( 'NONE', *, *, #73274, .F. ) ;
#34814=CONICAL_SURFACE ( 'NONE', #105897, 0.09999999999999982514, 0.003490658503988666988 ) ;
#34815=ORIENTED_EDGE ( 'NONE', *, *, #90454, .F. ) ;
#34816=DIRECTION ( 'NONE',  ( 0.000000000000000000, 1.000000000000000000, 0.000000000000000000 ) ) ;
#34817=DIRECTION ( 'NONE',  ( -0.000000000000000000, 1.000000000000000000, -0.000000000000000000 ) ) ;
#34818=LINE ( 'NONE', #63619, #124490 ) ;
#34819=CARTESIAN_POINT ( 'NONE',  ( -5.400000000000019895, 2.500000000000000000, -0.6928203230275541413 ) ) ;
#34820=EDGE_LOOP ( 'NONE', ( #73945, #96470, #101607, #105504 ) ) ;
#34821=VERTEX_POINT ( 'NONE', #112534 ) ;
#34822=PLANE ( 'NONE',  #64137 ) ;
#34823=EDGE_LOOP ( 'NONE', ( #108751, #37435, #37161, #23733 ) ) ;
#34824=CARTESIAN_POINT ( 'NONE',  ( -10.65000000000000213, 2.500000000000000000, 2.411473670974873862 ) ) ;
#34825=DIRECTION ( 'NONE',  ( 0.000000000000000000, 0.000000000000000000, 1.000000000000000000 ) ) ;
#34826=CIRCLE ( 'NONE', #43234, 0.06509327318403745899 ) ;
#34827=EDGE_LOOP ( 'NONE', ( #56802, #328 ) ) ;
#34829=LINE ( 'NONE', #66821, #22310 ) ;
#34830=CARTESIAN_POINT ( 'NONE',  ( -3.950000000000024603, 2.500000000000000000, -2.511473670974877948 ) ) ;
#34831=AXIS2_PLACEMENT_3D ( 'NONE', #54153, #23384, #103255 ) ;
#34832=AXIS2_PLACEMENT_3D ( 'NONE', #26917, #87116, #84547 ) ;
#34833=DIRECTION ( 'NONE',  ( -0.000000000000000000, -1.000000000000000000, -0.000000000000000000 ) ) ;
#34834=DIRECTION ( 'NONE',  ( -0.000000000000000000, 1.000000000000000000, -0.000000000000000000 ) ) ;
#34835=CARTESIAN_POINT ( 'NONE',  ( 0.6499999999999543920, 2.500000000000000000, 6.941600689897073018 ) ) ;
#34837=DIRECTION ( 'NONE',  ( 0.000000000000000000, -0.000000000000000000, 1.000000000000000000 ) ) ;
#34838=DIRECTION ( 'NONE',  ( 0.000000000000000000, 0.000000000000000000, 1.000000000000000000 ) ) ;
#34839=ORIENTED_EDGE ( 'NONE', *, *, #64170, .F. ) ;
#34840=EDGE_LOOP ( 'NONE', ( #39881, #57995, #7999, #76059 ) ) ;
#34841=ORIENTED_EDGE ( 'NONE', *, *, #16745, .F. ) ;
#34842=DIRECTION ( 'NONE',  ( 0.000000000000000000, -0.9999939076577903929, 0.003490651415223739937 ) ) ;
#34843=ORIENTED_EDGE ( 'NONE', *, *, #129130, .T. ) ;
#34844=DIRECTION ( 'NONE',  ( 0.000000000000000000, 0.000000000000000000, -1.000000000000000000 ) ) ;
#34845=ORIENTED_EDGE ( 'NONE', *, *, #41322, .F. ) ;
#34846=EDGE_LOOP ( 'NONE', ( #3163, #34534 ) ) ;
#34847=EDGE_LOOP ( 'NONE', ( #63196, #32845 ) ) ;
#34848=DIRECTION ( 'NONE',  ( 0.000000000000000000, 0.000000000000000000, 1.000000000000000000 ) ) ;
#34849=LINE ( 'NONE', #36777, #61510 ) ;
#34850=DIRECTION ( 'NONE',  ( 0.000000000000000000, 1.000000000000000000, 0.000000000000000000 ) ) ;
#34851=CARTESIAN_POINT ( 'NONE',  ( -3.642919299551294898E-14, 2.500000000000000000, 0.7928203230275517877 ) ) ;
#34852=CARTESIAN_POINT ( 'NONE',  ( -9.350000000000008527, 2.500000000000000000, -6.841600689897072485 ) ) ;
#34853=ORIENTED_EDGE ( 'NONE', *, *, #3386, .F. ) ;
#34854=EDGE_CURVE ( 'NONE', #103956, #123894, #38380, .T. ) ;
#34855=FACE_OUTER_BOUND ( 'NONE', #127124, .T. ) ;
#34856=ORIENTED_EDGE ( 'NONE', *, *, #5681, .T. ) ;
#34857=EDGE_CURVE ( 'NONE', #36092, #62518, #13208, .T. ) ;
#34858=AXIS2_PLACEMENT_3D ( 'NONE', #54294, #44470, #5177 ) ;
#34859=ORIENTED_EDGE ( 'NONE', *, *, #42957, .F. ) ;
#34860=ORIENTED_EDGE ( 'NONE', *, *, #88745, .F. ) ;
#34861=AXIS2_PLACEMENT_3D ( 'NONE', #48404, #29418, #59550 ) ;
#34862=EDGE_CURVE ( 'NONE', #15846, #103155, #19477, .T. ) ;
#34863=LINE ( 'NONE', #125157, #92371 ) ;
#34864=EDGE_LOOP ( 'NONE', ( #118541, #5302 ) ) ;
#34865=ORIENTED_EDGE ( 'NONE', *, *, #57078, .F. ) ;
#34866=VERTEX_POINT ( 'NONE', #111881 ) ;
#34867=PLANE ( 'NONE',  #111409 ) ;
#34868=ADVANCED_FACE ( 'NONE', ( #22226 ), #101053, .T. ) ;
#34869=CIRCLE ( 'NONE', #87060, 0.06509327318403745899 ) ;
#34870=CONICAL_SURFACE ( 'NONE', #43273, 0.1000000000000002554, 0.003490658503988666988 ) ;
#34871=CARTESIAN_POINT ( 'NONE',  ( 4.149999999999941735, 2.500000000000000000, -2.857883832488653741 ) ) ;
#34872=FACE_OUTER_BOUND ( 'NONE', #82016, .T. ) ;
#34873=CARTESIAN_POINT ( 'NONE',  ( 3.349999999999945466, 2.500000000000000000, -2.065063509461102065 ) ) ;
#34874=CARTESIAN_POINT ( 'NONE',  ( -12.69999999999999041, 2.500000000000000000, 3.983716857408420964 ) ) ;
#34875=CARTESIAN_POINT ( 'NONE',  ( 3.349999999999941913, 2.500000000000000000, 6.595190528383296780 ) ) ;
#34877=DIRECTION ( 'NONE',  ( 0.000000000000000000, 0.000000000000000000, 1.000000000000000000 ) ) ;
#34878=AXIS2_PLACEMENT_3D ( 'NONE', #30227, #70142, #73337 ) ;
#34879=AXIS2_PLACEMENT_3D ( 'NONE', #54394, #26238, #114597 ) ;
#34880=ORIENTED_EDGE ( 'NONE', *, *, #11933, .T. ) ;
#34881=CARTESIAN_POINT ( 'NONE',  ( -7.100000000000017408, 2.500000000000000000, 0.5928203230275495006 ) ) ;
#34882=CIRCLE ( 'NONE', #22260, 0.1000000000000002554 ) ;
#34883=ORIENTED_EDGE ( 'NONE', *, *, #37237, .F. ) ;
#34884=CARTESIAN_POINT ( 'NONE',  ( 1.899999999999951283, 12.50000000000000000, -3.918623584224389056 ) ) ;
#34885=ORIENTED_EDGE ( 'NONE', *, *, #124796, .T. ) ;
#34886=ADVANCED_FACE ( 'NONE', ( #16226 ), #61353, .T. ) ;
#34887=ORIENTED_EDGE ( 'NONE', *, *, #23727, .F. ) ;
#34888=DIRECTION ( 'NONE',  ( 0.000000000000000000, 0.000000000000000000, 1.000000000000000000 ) ) ;
#34889=CARTESIAN_POINT ( 'NONE',  ( -10.84999999999999964, 2.500000000000000000, 2.857883832488649301 ) ) ;
#34890=CARTESIAN_POINT ( 'NONE',  ( -11.89999999999999680, 2.500000000000000000, -0.3464101615137741841 ) ) ;
#34891=DIRECTION ( 'NONE',  ( 0.000000000000000000, 0.000000000000000000, -1.000000000000000000 ) ) ;
#34892=ORIENTED_EDGE ( 'NONE', *, *, #48549, .F. ) ;
#34893=LINE ( 'NONE', #65613, #81210 ) ;
#34894=DIRECTION ( 'NONE',  ( -0.000000000000000000, 1.000000000000000000, -0.000000000000000000 ) ) ;
#34895=LINE ( 'NONE', #73495, #125422 ) ;
#34896=AXIS2_PLACEMENT_3D ( 'NONE', #119479, #79575, #9546 ) ;
#34897=CARTESIAN_POINT ( 'NONE',  ( 9.549999999999918998, 12.50000000000000000, 2.165063509461097713 ) ) ;
#34898=CIRCLE ( 'NONE', #28621, 0.09999999999999982514 ) ;
#34899=CARTESIAN_POINT ( 'NONE',  ( 3.099999999999945022, 12.50000000000000000, -4.611443907251940644 ) ) ;
#34900=EDGE_LOOP ( 'NONE', ( #71199, #11477 ) ) ;
#34901=AXIS2_PLACEMENT_3D ( 'NONE', #13328, #33635, #102377 ) ;
#34902=EDGE_CURVE ( 'NONE', #107815, #125293, #85631, .T. ) ;
#34903=ORIENTED_EDGE ( 'NONE', *, *, #33018, .T. ) ;
#34904=AXIS2_PLACEMENT_3D ( 'NONE', #3086, #33818, #84852 ) ;
#34905=ORIENTED_EDGE ( 'NONE', *, *, #14223, .T. ) ;
#34906=CONICAL_SURFACE ( 'NONE', #120562, 0.1000000000000000056, 0.003490658503988666988 ) ;
#34907=DIRECTION ( 'NONE',  ( 0.000000000000000000, 0.000000000000000000, 1.000000000000000000 ) ) ;
#34908=CARTESIAN_POINT ( 'NONE',  ( 17.50000000000000000, 2.500000000000000000, -3.999999999999996447 ) ) ;
#34909=CIRCLE ( 'NONE', #11890, 0.1000000000000000472 ) ;
#34911=CARTESIAN_POINT ( 'NONE',  ( 9.149999999999920419, 2.500000000000000000, 1.472243186433545459 ) ) ;
#34912=AXIS2_PLACEMENT_3D ( 'NONE', #26136, #16285, #54298 ) ;
#34913=FACE_OUTER_BOUND ( 'NONE', #6509, .T. ) ;
#34915=DIRECTION ( 'NONE',  ( 0.000000000000000000, -0.9999939076577903929, 0.003490651415223739937 ) ) ;
#34916=FACE_OUTER_BOUND ( 'NONE', #103844, .T. ) ;
#34918=VECTOR ( 'NONE', #31550, 1000.000000000000000 ) ;
#34920=AXIS2_PLACEMENT_3D ( 'NONE', #94211, #84390, #64744 ) ;
#34921=CARTESIAN_POINT ( 'NONE',  ( 2.299999999999948752, 2.500000000000000000, -4.083716857408426826 ) ) ;
#34922=DIRECTION ( 'NONE',  ( -0.000000000000000000, -1.000000000000000000, -0.000000000000000000 ) ) ;
#34923=ORIENTED_EDGE ( 'NONE', *, *, #72324, .F. ) ;
#34924=EDGE_CURVE ( 'NONE', #55864, #50530, #126082, .T. ) ;
#34925=CARTESIAN_POINT ( 'NONE',  ( -9.600000000000006750, 12.50000000000000000, 5.088040615133786027 ) ) ;
#34926=VERTEX_POINT ( 'NONE', #65991 ) ;
#34927=DIRECTION ( 'NONE',  ( -4.274815082592931898E-19, -0.9999939076577903929, -0.003490651415223739937 ) ) ;
#34928=EDGE_LOOP ( 'NONE', ( #53208, #104309, #93293, #47336 ) ) ;
#34929=DIRECTION ( 'NONE',  ( 0.000000000000000000, -0.9999939076577903929, 0.003490651415223739937 ) ) ;
#34930=FACE_OUTER_BOUND ( 'NONE', #40314, .T. ) ;
#34931=VECTOR ( 'NONE', #17405, 1000.000000000000000 ) ;
#34932=CARTESIAN_POINT ( 'NONE',  ( -9.400000000000007461, 2.500000000000000000, -0.3464101615137783474 ) ) ;
#34934=DIRECTION ( 'NONE',  ( 0.000000000000000000, 0.000000000000000000, -1.000000000000000000 ) ) ;
#34935=ADVANCED_FACE ( 'NONE', ( #46346 ), #59314, .T. ) ;
#34936=DIRECTION ( 'NONE',  ( 0.000000000000000000, 0.000000000000000000, -1.000000000000000000 ) ) ;
#34937=ORIENTED_EDGE ( 'NONE', *, *, #86961, .F. ) ;
#34938=CARTESIAN_POINT ( 'NONE',  ( 10.64999999999990976, 2.500000000000000000, -6.741600689897077281 ) ) ;
#34939=EDGE_CURVE ( 'NONE', #121018, #3070, #55084, .T. ) ;
#34940=VECTOR ( 'NONE', #42399, 1000.000000000000000 ) ;
#34941=ORIENTED_EDGE ( 'NONE', *, *, #6803, .F. ) ;
#34942=ORIENTED_EDGE ( 'NONE', *, *, #101543, .T. ) ;
#34943=DIRECTION ( 'NONE',  ( 0.000000000000000000, 0.000000000000000000, 1.000000000000000000 ) ) ;
#34944=DIRECTION ( 'NONE',  ( 0.000000000000000000, 1.000000000000000000, 0.000000000000000000 ) ) ;
#34945=ADVANCED_FACE ( 'NONE', ( #64700 ), #128260, .T. ) ;
#34946=EDGE_CURVE ( 'NONE', #71349, #80664, #6934, .T. ) ;
#34947=EDGE_LOOP ( 'NONE', ( #101959, #13696 ) ) ;
#34948=EDGE_CURVE ( 'NONE', #43610, #27804, #126206, .T. ) ;
#34949=EDGE_CURVE ( 'NONE', #61414, #70903, #6394, .T. ) ;
#34950=FACE_OUTER_BOUND ( 'NONE', #125029, .T. ) ;
#34951=CARTESIAN_POINT ( 'NONE',  ( -13.09999999999999254, 12.50000000000000000, -0.4115034346978115321 ) ) ;
#34952=ORIENTED_EDGE ( 'NONE', *, *, #87778, .T. ) ;
#34953=AXIS2_PLACEMENT_3D ( 'NONE', #75295, #25534, #105411 ) ;
#34954=DIRECTION ( 'NONE',  ( -0.000000000000000000, -1.000000000000000000, -0.000000000000000000 ) ) ;
#34955=CARTESIAN_POINT ( 'NONE',  ( -9.150000000000005684, 12.50000000000000000, 5.802370205355744659 ) ) ;
#34956=EDGE_CURVE ( 'NONE', #27189, #74312, #103108, .T. ) ;
#34957=DIRECTION ( 'NONE',  ( 0.000000000000000000, 0.000000000000000000, 1.000000000000000000 ) ) ;
#34958=FACE_OUTER_BOUND ( 'NONE', #10380, .T. ) ;
#34959=CARTESIAN_POINT ( 'NONE',  ( 5.799999999999934985, 2.500000000000000000, -4.330127018922201643 ) ) ;
#34960=EDGE_CURVE ( 'NONE', #92950, #60183, #34626, .T. ) ;
#34961=LINE ( 'NONE', #75494, #36775 ) ;
#34962=DIRECTION ( 'NONE',  ( -0.000000000000000000, 1.000000000000000000, -0.000000000000000000 ) ) ;
#34963=ADVANCED_FACE ( 'NONE', ( #74531 ), #96835, .T. ) ;
#34964=VECTOR ( 'NONE', #105052, 1000.000000000000000 ) ;
#34965=AXIS2_PLACEMENT_3D ( 'NONE', #128821, #79059, #86264 ) ;
#34966=EDGE_CURVE ( 'NONE', #12963, #122201, #23691, .T. ) ;
#34967=CIRCLE ( 'NONE', #1489, 0.06509327318403745899 ) ;
#34968=EDGE_CURVE ( 'NONE', #123444, #69018, #57231, .T. ) ;
#34969=VERTEX_POINT ( 'NONE', #115731 ) ;
#34970=VERTEX_POINT ( 'NONE', #5133 ) ;
#34972=EDGE_LOOP ( 'NONE', ( #34201, #30512 ) ) ;
#34973=DIRECTION ( 'NONE',  ( 0.000000000000000000, -0.000000000000000000, 1.000000000000000000 ) ) ;
#34974=DIRECTION ( 'NONE',  ( 0.000000000000000000, 0.000000000000000000, -1.000000000000000000 ) ) ;
#34975=DIRECTION ( 'NONE',  ( 0.000000000000000000, -0.9999939076577903929, 0.003490651415223739937 ) ) ;
#34976=VERTEX_POINT ( 'NONE', #65334 ) ;
#34977=ADVANCED_FACE ( 'NONE', ( #45083 ), #69751, .T. ) ;
#34978=FACE_BOUND ( 'NONE', #34067, .T. ) ;
#34980=CARTESIAN_POINT ( 'NONE',  ( -12.29999999999999538, 12.50000000000000000, -0.4115034346978116431 ) ) ;
#34981=CARTESIAN_POINT ( 'NONE',  ( 10.79999999999991012, 12.50000000000000000, -4.330127018922201643 ) ) ;
#34982=CARTESIAN_POINT ( 'NONE',  ( 11.64999999999990443, 2.500000000000000000, -7.288010851410854585 ) ) ;
#34983=CARTESIAN_POINT ( 'NONE',  ( -15.39999999999998082, 2.500000000000000000, 0.7928203230275517877 ) ) ;
#34984=CARTESIAN_POINT ( 'NONE',  ( 7.099999999999928590, 12.50000000000000000, -4.957854068765716882 ) ) ;
#34985=CARTESIAN_POINT ( 'NONE',  ( 4.999999999999973355, 2.500000000000000000, -4.230127018922201998 ) ) ;
#34986=DIRECTION ( 'NONE',  ( -0.000000000000000000, -1.000000000000000000, -0.000000000000000000 ) ) ;
#34987=DIRECTION ( 'NONE',  ( 0.000000000000000000, 1.000000000000000000, 0.000000000000000000 ) ) ;
#34988=CARTESIAN_POINT ( 'NONE',  ( 5.849999999999932143, 12.50000000000000000, 2.099970236277060032 ) ) ;
#34989=CONICAL_SURFACE ( 'NONE', #39196, 0.1000000000000000056, 0.003490658503988666988 ) ;
#34990=AXIS2_PLACEMENT_3D ( 'NONE', #64899, #23705, #43999 ) ;
#34991=FACE_OUTER_BOUND ( 'NONE', #59978, .T. ) ;
#34992=ORIENTED_EDGE ( 'NONE', *, *, #29238, .F. ) ;
#34993=AXIS2_PLACEMENT_3D ( 'NONE', #71613, #101079, #2216 ) ;
#34994=ORIENTED_EDGE ( 'NONE', *, *, #29022, .F. ) ;
#34995=ORIENTED_EDGE ( 'NONE', *, *, #92327, .T. ) ;
#34996=ORIENTED_EDGE ( 'NONE', *, *, #5883, .T. ) ;
#34997=CARTESIAN_POINT ( 'NONE',  ( -3.100000000000028511, 12.50000000000000000, -0.3464101615137782364 ) ) ;
#34998=ORIENTED_EDGE ( 'NONE', *, *, #94317, .F. ) ;
#34999=CARTESIAN_POINT ( 'NONE',  ( -9.400000000000009237, 12.50000000000000000, -3.983716857408421852 ) ) ;
#35000=ORIENTED_EDGE ( 'NONE', *, *, #1550, .T. ) ;
#35001=AXIS2_PLACEMENT_3D ( 'NONE', #4834, #33051, #44794 ) ;
#35002=ORIENTED_EDGE ( 'NONE', *, *, #52578, .F. ) ;
#35003=AXIS2_PLACEMENT_3D ( 'NONE', #41737, #33203, #31901 ) ;
#35004=AXIS2_PLACEMENT_3D ( 'NONE', #70282, #89268, #109558 ) ;
#35005=VECTOR ( 'NONE', #8478, 1000.000000000000000 ) ;
#35006=FACE_OUTER_BOUND ( 'NONE', #23977, .T. ) ;
#35007=DIRECTION ( 'NONE',  ( -0.000000000000000000, 1.000000000000000000, -0.000000000000000000 ) ) ;
#35008=CARTESIAN_POINT ( 'NONE',  ( -14.34999999999998543, 2.500000000000000000, -1.718653347947323606 ) ) ;
#35009=DIRECTION ( 'NONE',  ( 0.000000000000000000, 1.000000000000000000, 0.000000000000000000 ) ) ;
#35010=AXIS2_PLACEMENT_3D ( 'NONE', #71864, #101324, #63318 ) ;
#35011=ORIENTED_EDGE ( 'NONE', *, *, #64631, .F. ) ;
#35012=ORIENTED_EDGE ( 'NONE', *, *, #47225, .T. ) ;
#35013=ADVANCED_FACE ( 'NONE', ( #28662 ), #70500, .T. ) ;
#35014=AXIS2_PLACEMENT_3D ( 'NONE', #4230, #56556, #116771 ) ;
#35015=VECTOR ( 'NONE', #38016, 1000.000000000000000 ) ;
#35016=EDGE_LOOP ( 'NONE', ( #38875, #82640 ) ) ;
#35017=DIRECTION ( 'NONE',  ( 0.000000000000000000, 1.000000000000000000, 0.000000000000000000 ) ) ;
#35018=ORIENTED_EDGE ( 'NONE', *, *, #103481, .F. ) ;
#35019=ADVANCED_FACE ( 'NONE', ( #100598 ), #8352, .T. ) ;
#35020=DIRECTION ( 'NONE',  ( -4.274815082592931898E-19, -0.9999939076577903929, -0.003490651415223739937 ) ) ;
#35021=EDGE_LOOP ( 'NONE', ( #13384, #39042, #121222, #28762 ) ) ;
#35022=ORIENTED_EDGE ( 'NONE', *, *, #28365, .F. ) ;
#35023=DIRECTION ( 'NONE',  ( 0.000000000000000000, 0.000000000000000000, -1.000000000000000000 ) ) ;
#35024=EDGE_CURVE ( 'NONE', #78315, #121706, #103201, .T. ) ;
#35025=DIRECTION ( 'NONE',  ( -0.000000000000000000, -1.000000000000000000, -0.000000000000000000 ) ) ;
#35026=DIRECTION ( 'NONE',  ( -0.000000000000000000, -1.000000000000000000, -0.000000000000000000 ) ) ;
#35027=CARTESIAN_POINT ( 'NONE',  ( 12.09999999999990195, 12.50000000000000000, -0.6277270498435166823 ) ) ;
#35028=DIRECTION ( 'NONE',  ( 0.000000000000000000, 1.000000000000000000, 0.000000000000000000 ) ) ;
#35029=AXIS2_PLACEMENT_3D ( 'NONE', #39038, #29834, #128710 ) ;
#35030=VERTEX_POINT ( 'NONE', #109794 ) ;
#35031=CARTESIAN_POINT ( 'NONE',  ( 0.3999999999999563904, 2.500000000000000000, 4.922947341949748257 ) ) ;
#35032=EDGE_LOOP ( 'NONE', ( #56492, #49700, #115985, #104480 ) ) ;
#35033=CARTESIAN_POINT ( 'NONE',  ( -5.850000000000018296, 12.50000000000000000, 5.802370205355744659 ) ) ;
#35034=EDGE_LOOP ( 'NONE', ( #16991, #45070 ) ) ;
#35035=CARTESIAN_POINT ( 'NONE',  ( -1.250000000000001110, 12.50000000000000000, -6.430097255199264339 ) ) ;
#35036=DIRECTION ( 'NONE',  ( -0.000000000000000000, -1.000000000000000000, -0.000000000000000000 ) ) ;
#35037=DIRECTION ( 'NONE',  ( 0.000000000000000000, 1.000000000000000000, 0.000000000000000000 ) ) ;
#35038=DIRECTION ( 'NONE',  ( 0.000000000000000000, 1.000000000000000000, 0.000000000000000000 ) ) ;
#35039=ORIENTED_EDGE ( 'NONE', *, *, #63070, .F. ) ;
#35040=( NAMED_UNIT ( * ) PLANE_ANGLE_UNIT ( ) SI_UNIT ( $, .RADIAN. ) );
#35041=AXIS2_PLACEMENT_3D ( 'NONE', #42086, #53202, #100992 ) ;
#35043=DIRECTION ( 'NONE',  ( -0.000000000000000000, -1.000000000000000000, -0.000000000000000000 ) ) ;
#35044=EDGE_LOOP ( 'NONE', ( #98133, #107711 ) ) ;
#35045=ORIENTED_EDGE ( 'NONE', *, *, #117738, .T. ) ;
#35046=ORIENTED_EDGE ( 'NONE', *, *, #39686, .F. ) ;
#35047=DIRECTION ( 'NONE',  ( 0.000000000000000000, 0.000000000000000000, 1.000000000000000000 ) ) ;
#35048=DIRECTION ( 'NONE',  ( 0.000000000000000000, 0.000000000000000000, 1.000000000000000000 ) ) ;
#35050=DIRECTION ( 'NONE',  ( -4.274815082592931898E-19, -0.9999939076577903929, -0.003490651415223739937 ) ) ;
#35051=CONICAL_SURFACE ( 'NONE', #5755, 0.1000000000000002554, 0.003490658503988666988 ) ;
#35052=AXIS2_PLACEMENT_3D ( 'NONE', #86874, #105230, #56747 ) ;
#35053=EDGE_CURVE ( 'NONE', #16096, #29908, #69201, .T. ) ;
#35054=AXIS2_PLACEMENT_3D ( 'NONE', #60451, #42084, #80723 ) ;
#35055=CARTESIAN_POINT ( 'NONE',  ( -7.100000000000017408, 12.50000000000000000, -0.6928203230275542523 ) ) ;
#35056=DIRECTION ( 'NONE',  ( 0.000000000000000000, 0.000000000000000000, -1.000000000000000000 ) ) ;
#35057=EDGE_LOOP ( 'NONE', ( #111986, #44497 ) ) ;
#35058=CARTESIAN_POINT ( 'NONE',  ( 105.5000000000000142, 0.000000000000000000, 0.000000000000000000 ) ) ;
#35059=ORIENTED_EDGE ( 'NONE', *, *, #33883, .F. ) ;
#35060=EDGE_CURVE ( 'NONE', #47494, #31560, #13301, .T. ) ;
#35061=FACE_OUTER_BOUND ( 'NONE', #125821, .T. ) ;
#35062=PLANE ( 'NONE',  #86070 ) ;
#35063=EDGE_CURVE ( 'NONE', #35289, #104203, #101152, .T. ) ;
#35064=CARTESIAN_POINT ( 'NONE',  ( 2.699999999999946443, 12.50000000000000000, 0.3464101615137735735 ) ) ;
#35066=VECTOR ( 'NONE', #60579, 1000.000000000000000 ) ;
#35067=CARTESIAN_POINT ( 'NONE',  ( -3.749999999999991562, 2.500000000000000000, 6.495190528383297135 ) ) ;
#35068=DIRECTION ( 'NONE',  ( -0.000000000000000000, -1.000000000000000000, -0.000000000000000000 ) ) ;
#35069=VECTOR ( 'NONE', #36755, 1000.000000000000000 ) ;
#35071=AXIS2_PLACEMENT_3D ( 'NONE', #62034, #44816, #124662 ) ;
#35073=CONICAL_SURFACE ( 'NONE', #106068, 0.1000000000000002554, 0.003490658503988666988 ) ;
#35074=CARTESIAN_POINT ( 'NONE',  ( -4.400000000000025224, 2.500000000000000000, 0.4464101615137735513 ) ) ;
#35075=VECTOR ( 'NONE', #108295, 1000.000000000000000 ) ;
#35076=ORIENTED_EDGE ( 'NONE', *, *, #127563, .T. ) ;
#35077=ORIENTED_EDGE ( 'NONE', *, *, #113831, .F. ) ;
#35078=CARTESIAN_POINT ( 'NONE',  ( -0.2000000000000347888, 12.50000000000000000, 0.3464101615137758494 ) ) ;
#35079=VECTOR ( 'NONE', #40789, 1000.000000000000000 ) ;
#35080=VERTEX_POINT ( 'NONE', #48948 ) ;
#35081=CARTESIAN_POINT ( 'NONE',  ( 5.199999999999935341, 12.50000000000000000, -0.4115034346978157509 ) ) ;
#35082=DIRECTION ( 'NONE',  ( 0.000000000000000000, 0.000000000000000000, -1.000000000000000000 ) ) ;
#35083=DIRECTION ( 'NONE',  ( -0.000000000000000000, -1.000000000000000000, -0.000000000000000000 ) ) ;
#35084=EDGE_LOOP ( 'NONE', ( #10122, #43701 ) ) ;
#35085=CONICAL_SURFACE ( 'NONE', #76928, 0.1000000000000002554, 0.003490658503988666988 ) ;
#35086=FACE_BOUND ( 'NONE', #67955, .T. ) ;
#35087=CARTESIAN_POINT ( 'NONE',  ( 6.899999999999928413, 12.50000000000000000, 4.676537180435972552 ) ) ;
#35088=CARTESIAN_POINT ( 'NONE',  ( 13.09999999999990195, 2.500000000000000000, 4.676537180435972552 ) ) ;
#35089=ORIENTED_EDGE ( 'NONE', *, *, #15100, .F. ) ;
#35090=DIRECTION ( 'NONE',  ( -0.000000000000000000, -1.000000000000000000, -0.000000000000000000 ) ) ;
#35091=CIRCLE ( 'NONE', #106187, 0.1000000000000000472 ) ;
#35093=EDGE_LOOP ( 'NONE', ( #15173, #9471, #46990, #45488 ) ) ;
#35094=EDGE_CURVE ( 'NONE', #93190, #73490, #36329, .T. ) ;
#35096=CONICAL_SURFACE ( 'NONE', #26764, 0.09999999999999999167, 0.003490658503988666988 ) ;
#35097=ORIENTED_EDGE ( 'NONE', *, *, #77597, .F. ) ;
#35098=VERTEX_POINT ( 'NONE', #47655 ) ;
#35099=DIRECTION ( 'NONE',  ( 0.000000000000000000, 0.000000000000000000, 1.000000000000000000 ) ) ;
#35100=CARTESIAN_POINT ( 'NONE',  ( -10.84999999999999964, 12.50000000000000000, 2.857883832488649301 ) ) ;
#35101=LINE ( 'NONE', #85465, #35776 ) ;
#35102=EDGE_CURVE ( 'NONE', #79548, #82957, #46781, .T. ) ;
#35103=FACE_BOUND ( 'NONE', #77428, .T. ) ;
#35104=ORIENTED_EDGE ( 'NONE', *, *, #79304, .F. ) ;
#35106=ADVANCED_FACE ( 'NONE', ( #110426 ), #87557, .T. ) ;
#35107=FACE_OUTER_BOUND ( 'NONE', #112379, .T. ) ;
#35108=CARTESIAN_POINT ( 'NONE',  ( 13.14999999999990088, 2.500000000000000000, 2.411473670974873862 ) ) ;
#35109=CARTESIAN_POINT ( 'NONE',  ( 12.09999999999990550, 2.500000000000000000, 4.230127018922196669 ) ) ;
#35110=ADVANCED_FACE ( 'NONE', ( #120264 ), #117847, .T. ) ;
#35112=EDGE_CURVE ( 'NONE', #20003, #55549, #119594, .T. ) ;
#35113=FACE_OUTER_BOUND ( 'NONE', #56829, .T. ) ;
#35114=EDGE_CURVE ( 'NONE', #93230, #8603, #86463, .T. ) ;
#35115=CARTESIAN_POINT ( 'NONE',  ( 9.599999999999914380, 12.50000000000000000, 4.330127018922196314 ) ) ;
#35116=DIRECTION ( 'NONE',  ( 0.000000000000000000, 0.000000000000000000, -1.000000000000000000 ) ) ;
#35117=CARTESIAN_POINT ( 'NONE',  ( 1.249999999999988898, 12.50000000000000000, -6.495190528383302464 ) ) ;
#35118=EDGE_CURVE ( 'NONE', #13136, #20444, #50989, .T. ) ;
#35119=ORIENTED_EDGE ( 'NONE', *, *, #105709, .F. ) ;
#35120=EDGE_LOOP ( 'NONE', ( #22052, #94714 ) ) ;
#35121=EDGE_LOOP ( 'NONE', ( #25972, #46352 ) ) ;
#35123=VERTEX_POINT ( 'NONE', #37825 ) ;
#35124=CARTESIAN_POINT ( 'NONE',  ( -7.100000000000017408, 2.500000000000000000, -3.637306695894650055 ) ) ;
#35125=AXIS2_PLACEMENT_3D ( 'NONE', #1149, #111755, #51558 ) ;
#35126=CARTESIAN_POINT ( 'NONE',  ( 12.04999999999990834, 2.500000000000000000, 6.395190528383296602 ) ) ;
#35127=ORIENTED_EDGE ( 'NONE', *, *, #108689, .F. ) ;
#35128=FACE_BOUND ( 'NONE', #80837, .T. ) ;
#35129=ADVANCED_FACE ( 'NONE', ( #90124 ), #67687, .T. ) ;
#35130=CARTESIAN_POINT ( 'NONE',  ( 11.04999999999990834, 2.500000000000000000, -6.741600689897077281 ) ) ;
#35131=CIRCLE ( 'NONE', #51839, 0.09999999999999982514 ) ;
#35132=CIRCLE ( 'NONE', #118732, 0.06509327318403745899 ) ;
#35133=DIRECTION ( 'NONE',  ( 0.000000000000000000, 0.000000000000000000, 1.000000000000000000 ) ) ;
#35134=ORIENTED_EDGE ( 'NONE', *, *, #82421, .F. ) ;
#35135=DIRECTION ( 'NONE',  ( 0.000000000000000000, 0.000000000000000000, 1.000000000000000000 ) ) ;
#35137=CARTESIAN_POINT ( 'NONE',  ( -1.050000000000037348, 2.500000000000000000, -6.941600689897078347 ) ) ;
#35138=ORIENTED_EDGE ( 'NONE', *, *, #27418, .F. ) ;
#35139=CARTESIAN_POINT ( 'NONE',  ( 8.349999999999923261, 2.500000000000000000, -6.395190528383301931 ) ) ;
#35140=CONICAL_SURFACE ( 'NONE', #41395, 0.1000000000000002554, 0.003490658503988666988 ) ;
#35141=VERTEX_POINT ( 'NONE', #98662 ) ;
#35143=AXIS2_PLACEMENT_3D ( 'NONE', #107342, #80491, #122344 ) ;
#35144=ORIENTED_EDGE ( 'NONE', *, *, #44107, .T. ) ;
#35145=VERTEX_POINT ( 'NONE', #77729 ) ;
#35146=DIRECTION ( 'NONE',  ( -4.274815082592931898E-19, -0.9999939076577903929, -0.003490651415223739937 ) ) ;
#35148=DIRECTION ( 'NONE',  ( 0.000000000000000000, 0.000000000000000000, 1.000000000000000000 ) ) ;
#35149=VERTEX_POINT ( 'NONE', #117643 ) ;
#35150=CARTESIAN_POINT ( 'NONE',  ( 12.06068301313072411, 2.499999999999358735, -8.632776999393163564 ) ) ;
#35151=AXIS2_PLACEMENT_3D ( 'NONE', #125104, #55714, #43339 ) ;
#35152=LINE ( 'NONE', #95985, #44941 ) ;
#35153=CARTESIAN_POINT ( 'NONE',  ( 7.899999999999921307, 12.50000000000000000, 0.06509327318403504425 ) ) ;
#35155=CARTESIAN_POINT ( 'NONE',  ( -1.650000000000035660, 12.50000000000000000, 7.188010851410848723 ) ) ;
#35156=PLANE ( 'NONE',  #95556 ) ;
#35157=VERTEX_POINT ( 'NONE', #98028 ) ;
#35158=PLANE ( 'NONE',  #42079 ) ;
#35159=ORIENTED_EDGE ( 'NONE', *, *, #8944, .T. ) ;
#35160=EDGE_CURVE ( 'NONE', #10677, #62255, #124124, .T. ) ;
#35161=ORIENTED_EDGE ( 'NONE', *, *, #78347, .F. ) ;
#35162=FACE_OUTER_BOUND ( 'NONE', #93063, .T. ) ;
#35163=CARTESIAN_POINT ( 'NONE',  ( -11.84999999999999609, 2.500000000000000000, 6.841600689897072485 ) ) ;
#35164=FACE_OUTER_BOUND ( 'NONE', #51124, .T. ) ;
#35165=CARTESIAN_POINT ( 'NONE',  ( -4.350000000000023626, 12.50000000000000000, -2.511473670974877948 ) ) ;
#35166=DIRECTION ( 'NONE',  ( 0.000000000000000000, 1.000000000000000000, 0.000000000000000000 ) ) ;
#35167=ORIENTED_EDGE ( 'NONE', *, *, #37918, .T. ) ;
#35168=AXIS2_PLACEMENT_3D ( 'NONE', #62844, #61573, #31460 ) ;
#35169=ORIENTED_EDGE ( 'NONE', *, *, #30283, .T. ) ;
#35170=ADVANCED_FACE ( 'NONE', ( #122831 ), #61986, .T. ) ;
#35171=CARTESIAN_POINT ( 'NONE',  ( 15.19999999999989093, 2.500000000000000000, 0.2464101615137735679 ) ) ;
#35172=AXIS2_PLACEMENT_3D ( 'NONE', #97041, #49247, #127158 ) ;
#35173=CARTESIAN_POINT ( 'NONE',  ( 21.23528140090977345, 2.699413673072321718, -2.293764360948945757 ) ) ;
#35174=DIRECTION ( 'NONE',  ( -0.000000000000000000, -1.000000000000000000, -0.000000000000000000 ) ) ;
#35175=ORIENTED_EDGE ( 'NONE', *, *, #24588, .T. ) ;
#35176=ORIENTED_EDGE ( 'NONE', *, *, #98321, .T. ) ;
#35177=DIRECTION ( 'NONE',  ( -0.000000000000000000, 1.000000000000000000, -0.000000000000000000 ) ) ;
#35178=AXIS2_PLACEMENT_3D ( 'NONE', #104813, #127065, #15139 ) ;
#35179=ORIENTED_EDGE ( 'NONE', *, *, #28557, .T. ) ;
#35180=LINE ( 'NONE', #75086, #45769 ) ;
#35181=FACE_OUTER_BOUND ( 'NONE', #63388, .T. ) ;
#35182=ORIENTED_EDGE ( 'NONE', *, *, #78571, .F. ) ;
#35183=LINE ( 'NONE', #2461, #54417 ) ;
#35184=DIRECTION ( 'NONE',  ( 0.000000000000000000, 0.000000000000000000, -1.000000000000000000 ) ) ;
#35185=CARTESIAN_POINT ( 'NONE',  ( 12.09999999999990195, 2.500000000000000000, 0.7928203230275495672 ) ) ;
#35186=AXIS2_PLACEMENT_3D ( 'NONE', #34142, #2079, #31559 ) ;
#35188=ORIENTED_EDGE ( 'NONE', *, *, #107375, .T. ) ;
#35189=DIRECTION ( 'NONE',  ( 0.000000000000000000, 0.000000000000000000, 1.000000000000000000 ) ) ;
#35190=AXIS2_PLACEMENT_3D ( 'NONE', #117238, #67498, #97630 ) ;
#35191=VECTOR ( 'NONE', #31529, 1000.000000000000000 ) ;
#35192=DIRECTION ( 'NONE',  ( 0.000000000000000000, 0.000000000000000000, 1.000000000000000000 ) ) ;
#35193=ORIENTED_EDGE ( 'NONE', *, *, #29814, .F. ) ;
#35194=VERTEX_POINT ( 'NONE', #120888 ) ;
#35196=CARTESIAN_POINT ( 'NONE',  ( 4.549999999999937650, 2.500000000000000000, 2.265063509461097357 ) ) ;
#35197=CARTESIAN_POINT ( 'NONE',  ( -2.950000000000033484, 2.500000000000000000, -6.495190528383302464 ) ) ;
#35198=PLANE ( 'NONE',  #57457 ) ;
#35199=FACE_OUTER_BOUND ( 'NONE', #80853, .T. ) ;
#35200=EDGE_CURVE ( 'NONE', #111361, #128844, #63913, .T. ) ;
#35201=CYLINDRICAL_SURFACE ( 'NONE', #50940, 10.00000000000000000 ) ;
#35202=CARTESIAN_POINT ( 'NONE',  ( -14.54999999999998472, 2.500000000000000000, 2.165063509461101265 ) ) ;
#35203=DIRECTION ( 'NONE',  ( -0.000000000000000000, -1.000000000000000000, -0.000000000000000000 ) ) ;
#35204=CARTESIAN_POINT ( 'NONE',  ( -11.89999999999999680, 2.500000000000000000, -4.776537180435975749 ) ) ;
#35205=CARTESIAN_POINT ( 'NONE',  ( 4.199999999999938005, 2.500000000000000000, 4.330127018922196314 ) ) ;
#35206=ADVANCED_FACE ( 'NONE', ( #31241 ), #99104, .T. ) ;
#35207=VERTEX_POINT ( 'NONE', #82269 ) ;
#35208=VERTEX_POINT ( 'NONE', #113653 ) ;
#35209=CONICAL_SURFACE ( 'NONE', #28945, 0.09999999999999982514, 0.003490658503988666988 ) ;
#35210=ORIENTED_EDGE ( 'NONE', *, *, #55918, .F. ) ;
#35211=AXIS2_PLACEMENT_3D ( 'NONE', #9861, #51725, #1953 ) ;
#35212=VECTOR ( 'NONE', #89566, 1000.000000000000000 ) ;
#35213=EDGE_CURVE ( 'NONE', #97794, #61962, #80226, .T. ) ;
#35214=ORIENTED_EDGE ( 'NONE', *, *, #86096, .F. ) ;
#35215=PLANE ( 'NONE',  #123063 ) ;
#35216=EDGE_CURVE ( 'NONE', #122967, #46749, #73082, .T. ) ;
#35217=FACE_OUTER_BOUND ( 'NONE', #16346, .T. ) ;
#35218=CARTESIAN_POINT ( 'NONE',  ( -8.150000000000009237, 2.500000000000000000, 6.741600689897071952 ) ) ;
#35219=EDGE_LOOP ( 'NONE', ( #115291, #93257, #37292, #51669 ) ) ;
#35220=VECTOR ( 'NONE', #111282, 1000.000000000000000 ) ;
#35221=DIRECTION ( 'NONE',  ( 0.000000000000000000, 0.000000000000000000, 1.000000000000000000 ) ) ;
#35222=AXIS2_PLACEMENT_3D ( 'NONE', #41786, #123527, #1188 ) ;
#35223=EDGE_CURVE ( 'NONE', #6156, #52245, #63500, .T. ) ;
#35224=DIRECTION ( 'NONE',  ( 0.000000000000000000, 0.000000000000000000, 1.000000000000000000 ) ) ;
#35225=CARTESIAN_POINT ( 'NONE',  ( 8.349999999999923261, 12.50000000000000000, -6.495190528383302464 ) ) ;
#35226=VERTEX_POINT ( 'NONE', #72447 ) ;
#35228=CARTESIAN_POINT ( 'NONE',  ( -8.950000000000008171, 2.500000000000000000, 1.818653347947321475 ) ) ;
#35229=ORIENTED_EDGE ( 'NONE', *, *, #84326, .T. ) ;
#35230=AXIS2_PLACEMENT_3D ( 'NONE', #41961, #61608, #101520 ) ;
#35231=ORIENTED_EDGE ( 'NONE', *, *, #85313, .T. ) ;
#35232=VERTEX_POINT ( 'NONE', #101254 ) ;
#35233=ORIENTED_EDGE ( 'NONE', *, *, #89963, .F. ) ;
#35234=FACE_OUTER_BOUND ( 'NONE', #3451, .T. ) ;
#35235=DIRECTION ( 'NONE',  ( 0.000000000000000000, 0.000000000000000000, 1.000000000000000000 ) ) ;
#35236=CARTESIAN_POINT ( 'NONE',  ( -3.644143946350442628E-14, 2.500000000000000000, 0.5928203230275517210 ) ) ;
#35237=CARTESIAN_POINT ( 'NONE',  ( -2.050000000000033129, 2.500000000000000000, 2.165063509461097713 ) ) ;
#35238=EDGE_LOOP ( 'NONE', ( #126767, #83287 ) ) ;
#35239=DIRECTION ( 'NONE',  ( -0.000000000000000000, -1.000000000000000000, -0.000000000000000000 ) ) ;
#35240=ORIENTED_EDGE ( 'NONE', *, *, #58610, .F. ) ;
#35241=AXIS2_PLACEMENT_3D ( 'NONE', #45349, #85884, #114711 ) ;
#35242=CARTESIAN_POINT ( 'NONE',  ( 59.74180401167438959, -3.401974578012062267, -5.439313020133131005 ) ) ;
#35243=CARTESIAN_POINT ( 'NONE',  ( 10.84999999999990905, 2.500000000000000000, -6.495190528383302464 ) ) ;
#35245=CARTESIAN_POINT ( 'NONE',  ( -12.89999999999999147, 2.500000000000000000, -0.6928203230275500335 ) ) ;
#35246=EDGE_LOOP ( 'NONE', ( #5408, #54542 ) ) ;
#35247=ADVANCED_FACE ( 'NONE', ( #81608 ), #33801, .T. ) ;
#35249=ORIENTED_EDGE ( 'NONE', *, *, #82414, .F. ) ;
#35250=VERTEX_POINT ( 'NONE', #23989 ) ;
#35251=CARTESIAN_POINT ( 'NONE',  ( 13.29999999999989946, 2.500000000000000000, -2.385244779468109755E-15 ) ) ;
#35252=DIRECTION ( 'NONE',  ( 0.000000000000000000, 0.000000000000000000, 1.000000000000000000 ) ) ;
#35253=CARTESIAN_POINT ( 'NONE',  ( 2.499999999999948930, 2.500000000000000000, -5.022947341949754119 ) ) ;
#35254=FACE_BOUND ( 'NONE', #35034, .T. ) ;
#35255=CARTESIAN_POINT ( 'NONE',  ( -14.14999999999998614, 2.500000000000000000, -2.757883832488651876 ) ) ;
#35256=DIRECTION ( 'NONE',  ( 0.000000000000000000, 0.000000000000000000, 1.000000000000000000 ) ) ;
#35257=CONICAL_SURFACE ( 'NONE', #129359, 0.1000000000000000472, 0.003490658503988666988 ) ;
#35258=EDGE_CURVE ( 'NONE', #86589, #2147, #43013, .T. ) ;
#35259=DIRECTION ( 'NONE',  ( 0.000000000000000000, 0.000000000000000000, 1.000000000000000000 ) ) ;
#35260=VECTOR ( 'NONE', #31520, 1000.000000000000000 ) ;
#35261=EDGE_CURVE ( 'NONE', #129348, #84561, #1115, .T. ) ;
#35263=DIRECTION ( 'NONE',  ( 0.000000000000000000, 1.000000000000000000, 0.000000000000000000 ) ) ;
#35264=AXIS2_PLACEMENT_3D ( 'NONE', #29647, #110139, #109497 ) ;
#35265=ADVANCED_FACE ( 'NONE', ( #43642 ), #23791, .T. ) ;
#35266=PLANE ( 'NONE',  #3037 ) ;
#35267=ORIENTED_EDGE ( 'NONE', *, *, #103226, .F. ) ;
#35268=EDGE_CURVE ( 'NONE', #73774, #45181, #17504, .T. ) ;
#35269=DIRECTION ( 'NONE',  ( 0.000000000000000000, 1.000000000000000000, 0.000000000000000000 ) ) ;
#35270=CIRCLE ( 'NONE', #48074, 0.1000000000000002554 ) ;
#35271=EDGE_CURVE ( 'NONE', #14509, #113423, #61336, .T. ) ;
#35272=ORIENTED_EDGE ( 'NONE', *, *, #45150, .T. ) ;
#35273=VERTEX_POINT ( 'NONE', #123457 ) ;
#35274=VERTEX_POINT ( 'NONE', #91433 ) ;
#35275=ORIENTED_EDGE ( 'NONE', *, *, #72646, .T. ) ;
#35276=VECTOR ( 'NONE', #86116, 1000.000000000000000 ) ;
#35277=CARTESIAN_POINT ( 'NONE',  ( 4.349999999999940137, 12.50000000000000000, -6.841600689897078702 ) ) ;
#35278=FACE_BOUND ( 'NONE', #111773, .T. ) ;
#35279=PLANE ( 'NONE',  #70307 ) ;
#35280=ADVANCED_FACE ( 'NONE', ( #1752 ), #38472, .T. ) ;
#35281=CONICAL_SURFACE ( 'NONE', #3865, 0.1000000000000002554, 0.003490658503988666988 ) ;
#35282=EDGE_CURVE ( 'NONE', #82263, #103538, #4984, .T. ) ;
#35283=ORIENTED_EDGE ( 'NONE', *, *, #47531, .T. ) ;
#35284=DIRECTION ( 'NONE',  ( -0.000000000000000000, -1.000000000000000000, -0.000000000000000000 ) ) ;
#35285=DIRECTION ( 'NONE',  ( -0.000000000000000000, 1.000000000000000000, -0.000000000000000000 ) ) ;
#35286=ORIENTED_EDGE ( 'NONE', *, *, #123945, .T. ) ;
#35287=DIRECTION ( 'NONE',  ( -4.274815082592931898E-19, -0.9999939076577903929, -0.003490651415223739937 ) ) ;
#35288=CARTESIAN_POINT ( 'NONE',  ( 7.049999999999926992, 2.500000000000000000, 2.165063509461097713 ) ) ;
#35289=VERTEX_POINT ( 'NONE', #113005 ) ;
#35290=CIRCLE ( 'NONE', #95910, 0.1000000000000002554 ) ;
#35291=CARTESIAN_POINT ( 'NONE',  ( 11.24999999999994316, 2.500000000000000000, -6.495190528383302464 ) ) ;
#35292=CARTESIAN_POINT ( 'NONE',  ( -6.650000000000014566, 2.500000000000000000, 1.472243186433545459 ) ) ;
#35293=VERTEX_POINT ( 'NONE', #63260 ) ;
#35294=CIRCLE ( 'NONE', #41563, 0.06509327318403745899 ) ;
#35295=DIRECTION ( 'NONE',  ( 0.000000000000000000, 1.000000000000000000, 0.000000000000000000 ) ) ;
#35296=DIRECTION ( 'NONE',  ( 0.000000000000000000, 0.000000000000000000, -1.000000000000000000 ) ) ;
#35297=AXIS2_PLACEMENT_3D ( 'NONE', #63977, #103901, #15502 ) ;
#35298=DIRECTION ( 'NONE',  ( 0.000000000000000000, 0.000000000000000000, 1.000000000000000000 ) ) ;
#35299=VERTEX_POINT ( 'NONE', #115563 ) ;
#35300=EDGE_LOOP ( 'NONE', ( #128036, #23184 ) ) ;
#35301=DIRECTION ( 'NONE',  ( 0.000000000000000000, 0.000000000000000000, 1.000000000000000000 ) ) ;
#35302=AXIS2_PLACEMENT_3D ( 'NONE', #9442, #119378, #99761 ) ;
#35303=ORIENTED_EDGE ( 'NONE', *, *, #33531, .T. ) ;
#35304=CARTESIAN_POINT ( 'NONE',  ( 9.599999999999917932, 12.50000000000000000, -0.6277270498435166823 ) ) ;
#35305=FACE_OUTER_BOUND ( 'NONE', #86947, .T. ) ;
#35306=AXIS2_PLACEMENT_3D ( 'NONE', #67324, #37272, #126936 ) ;
#35307=AXIS2_PLACEMENT_3D ( 'NONE', #86830, #84248, #16137 ) ;
#35308=ORIENTED_EDGE ( 'NONE', *, *, #47085, .F. ) ;
#35309=CARTESIAN_POINT ( 'NONE',  ( 13.34999999999989662, 2.500000000000000000, -1.472243186433550122 ) ) ;
#35310=LINE ( 'NONE', #64748, #49786 ) ;
#35311=CARTESIAN_POINT ( 'NONE',  ( 10.84999999999991260, 2.500000000000000000, 6.595190528383296780 ) ) ;
#35312=CARTESIAN_POINT ( 'NONE',  ( -1.650000000000034772, 2.500000000000000000, 6.495190528383297135 ) ) ;
#35313=CARTESIAN_POINT ( 'NONE',  ( -0.4000000000000339950, 2.500000000000000000, 0.7928203230275517877 ) ) ;
#35314=VECTOR ( 'NONE', #30592, 1000.000000000000000 ) ;
#35315=ORIENTED_EDGE ( 'NONE', *, *, #66152, .T. ) ;
#35316=EDGE_CURVE ( 'NONE', #46102, #62111, #35740, .T. ) ;
#35317=CIRCLE ( 'NONE', #64639, 0.06509327318403741736 ) ;
#35318=ORIENTED_EDGE ( 'NONE', *, *, #126679, .F. ) ;
#35320=DIRECTION ( 'NONE',  ( 0.000000000000000000, 0.000000000000000000, 1.000000000000000000 ) ) ;
#35321=DIRECTION ( 'NONE',  ( 0.000000000000000000, -0.000000000000000000, 1.000000000000000000 ) ) ;
#35322=ORIENTED_EDGE ( 'NONE', *, *, #70510, .F. ) ;
#35323=ORIENTED_EDGE ( 'NONE', *, *, #125936, .F. ) ;
#35324=ORIENTED_EDGE ( 'NONE', *, *, #109075, .T. ) ;
#35325=CARTESIAN_POINT ( 'NONE',  ( 6.249999999999930722, 2.500000000000000000, 7.188010851410848723 ) ) ;
#35326=FACE_OUTER_BOUND ( 'NONE', #114303, .T. ) ;
#35327=CARTESIAN_POINT ( 'NONE',  ( -14.39999999999998614, 2.500000000000000000, 0.4464101615137758272 ) ) ;
#35328=DIRECTION ( 'NONE',  ( 0.000000000000000000, 0.000000000000000000, 1.000000000000000000 ) ) ;
#35329=LINE ( 'NONE', #123675, #104597 ) ;
#35330=FACE_OUTER_BOUND ( 'NONE', #11142, .T. ) ;
#35331=CARTESIAN_POINT ( 'NONE',  ( 11.44999999999991047, 2.500000000000000000, 6.148780366869520009 ) ) ;
#35332=AXIS2_PLACEMENT_3D ( 'NONE', #57421, #86864, #5718 ) ;
#35333=CARTESIAN_POINT ( 'NONE',  ( -0.6500000000000389910, 2.500000000000000000, -1.718653347947326049 ) ) ;
#35334=CARTESIAN_POINT ( 'NONE',  ( 6.849999999999927702, 2.500000000000000000, 2.411473670974873862 ) ) ;
#35335=ORIENTED_EDGE ( 'NONE', *, *, #99090, .F. ) ;
#35337=FACE_OUTER_BOUND ( 'NONE', #1943, .T. ) ;
#35338=EDGE_LOOP ( 'NONE', ( #47462, #64052, #112195, #96188 ) ) ;
#35339=VERTEX_POINT ( 'NONE', #25249 ) ;
#35340=CARTESIAN_POINT ( 'NONE',  ( 2.099999999999948574, 2.500000000000000000, 3.637306695894644726 ) ) ;
#35341=CARTESIAN_POINT ( 'NONE',  ( 10.84999999999990905, 12.50000000000000000, -7.188010851410854052 ) ) ;
#35342=CIRCLE ( 'NONE', #31150, 0.09999999999999999167 ) ;
#35343=DIRECTION ( 'NONE',  ( -0.000000000000000000, -1.000000000000000000, -0.000000000000000000 ) ) ;
#35344=CARTESIAN_POINT ( 'NONE',  ( 15.79999999999989058, 2.500000000000000000, -2.385244779468109755E-15 ) ) ;
#35345=CIRCLE ( 'NONE', #60399, 0.06509327318403745899 ) ;
#35346=DIRECTION ( 'NONE',  ( -0.000000000000000000, -1.000000000000000000, -0.000000000000000000 ) ) ;
#35347=PLANE ( 'NONE',  #57651 ) ;
#35348=CARTESIAN_POINT ( 'NONE',  ( 1.649999999999951505, 2.500000000000000000, -2.857883832488653741 ) ) ;
#35349=ORIENTED_EDGE ( 'NONE', *, *, #24438, .T. ) ;
#35350=FACE_OUTER_BOUND ( 'NONE', #39556, .T. ) ;
#35351=AXIS2_PLACEMENT_3D ( 'NONE', #124660, #35007, #6149 ) ;
#35352=DIRECTION ( 'NONE',  ( 0.000000000000000000, 1.000000000000000000, 0.000000000000000000 ) ) ;
#35353=ORIENTED_EDGE ( 'NONE', *, *, #87762, .T. ) ;
#35354=ADVANCED_FACE ( 'NONE', ( #35113 ), #116216, .T. ) ;
#35355=ORIENTED_EDGE ( 'NONE', *, *, #79761, .T. ) ;
#35356=VECTOR ( 'NONE', #12492, 1000.000000000000000 ) ;
#35357=CIRCLE ( 'NONE', #16454, 0.1000000000000002554 ) ;
#35358=EDGE_LOOP ( 'NONE', ( #84518, #95797, #108790, #99836 ) ) ;
#35359=ADVANCED_FACE ( 'NONE', ( #15429 ), #16710, .T. ) ;
#35360=ORIENTED_EDGE ( 'NONE', *, *, #86693, .F. ) ;
#35361=EDGE_CURVE ( 'NONE', #45135, #87037, #45569, .T. ) ;
#35362=FACE_OUTER_BOUND ( 'NONE', #21448, .T. ) ;
#35363=FACE_OUTER_BOUND ( 'NONE', #63344, .T. ) ;
#35364=AXIS2_PLACEMENT_3D ( 'NONE', #60674, #20096, #99303 ) ;
#35365=FACE_OUTER_BOUND ( 'NONE', #1682, .T. ) ;
#35366=PLANE ( 'NONE',  #111346 ) ;
#35367=EDGE_CURVE ( 'NONE', #26681, #87979, #30150, .T. ) ;
#35368=DIRECTION ( 'NONE',  ( 0.000000000000000000, 0.000000000000000000, 1.000000000000000000 ) ) ;
#35370=VERTEX_POINT ( 'NONE', #14146 ) ;
#35371=DIRECTION ( 'NONE',  ( -0.000000000000000000, 1.000000000000000000, -0.000000000000000000 ) ) ;
#35372=ADVANCED_FACE ( 'NONE', ( #54090 ), #124762, .T. ) ;
#35373=DIRECTION ( 'NONE',  ( 0.000000000000000000, 1.000000000000000000, 0.000000000000000000 ) ) ;
#35374=DIRECTION ( 'NONE',  ( 0.000000000000000000, -0.9999939076577903929, 0.003490651415223739937 ) ) ;
#35375=ORIENTED_EDGE ( 'NONE', *, *, #57580, .T. ) ;
#35376=ORIENTED_EDGE ( 'NONE', *, *, #104834, .T. ) ;
#35377=ORIENTED_EDGE ( 'NONE', *, *, #20346, .T. ) ;
#35378=CARTESIAN_POINT ( 'NONE',  ( 3.749999999999944045, 12.50000000000000000, -7.188010851410854052 ) ) ;
#35379=DIRECTION ( 'NONE',  ( -0.000000000000000000, 1.000000000000000000, -0.000000000000000000 ) ) ;
#35380=DIRECTION ( 'NONE',  ( 0.000000000000000000, 0.000000000000000000, 1.000000000000000000 ) ) ;
#35381=VECTOR ( 'NONE', #106519, 1000.000000000000000 ) ;
#35382=ORIENTED_EDGE ( 'NONE', *, *, #121357, .F. ) ;
#35383=DIRECTION ( 'NONE',  ( 0.000000000000000000, 1.000000000000000000, 0.000000000000000000 ) ) ;
#35384=DIRECTION ( 'NONE',  ( 0.000000000000000000, 1.000000000000000000, 0.000000000000000000 ) ) ;
#35385=DIRECTION ( 'NONE',  ( 0.000000000000000000, 0.000000000000000000, 1.000000000000000000 ) ) ;
#35386=DIRECTION ( 'NONE',  ( 0.000000000000000000, 0.000000000000000000, 1.000000000000000000 ) ) ;
#35387=CARTESIAN_POINT ( 'NONE',  ( 8.749999999999918288, 12.50000000000000000, 7.253104124594885960 ) ) ;
#35389=CONICAL_SURFACE ( 'NONE', #108543, 0.09999999999999982514, 0.003490658503988666988 ) ;
#35390=ORIENTED_EDGE ( 'NONE', *, *, #113084, .F. ) ;
#35391=AXIS2_PLACEMENT_3D ( 'NONE', #23553, #112595, #63487 ) ;
#35392=DIRECTION ( 'NONE',  ( 0.000000000000000000, 1.000000000000000000, 0.000000000000000000 ) ) ;
#35393=VERTEX_POINT ( 'NONE', #114925 ) ;
#35394=ORIENTED_EDGE ( 'NONE', *, *, #53522, .T. ) ;
#35395=VERTEX_POINT ( 'NONE', #94008 ) ;
#35396=ADVANCED_FACE ( 'NONE', ( #4969 ), #103302, .T. ) ;
#35397=CARTESIAN_POINT ( 'NONE',  ( 2.499999999999983569, 2.500000000000000000, 0.09999999999999772959 ) ) ;
#35398=FACE_BOUND ( 'NONE', #88386, .T. ) ;
#35399=CIRCLE ( 'NONE', #56307, 0.06509327318403745899 ) ;
#35400=CARTESIAN_POINT ( 'NONE',  ( 11.24999999999990941, 12.50000000000000000, 7.188010851410848723 ) ) ;
#35401=CARTESIAN_POINT ( 'NONE',  ( -8.150000000000009237, 2.500000000000000000, 6.148780366869520009 ) ) ;
#35402=CARTESIAN_POINT ( 'NONE',  ( 13.14999999999989733, 12.50000000000000000, -1.818653347947325916 ) ) ;
#35403=AXIS2_PLACEMENT_3D ( 'NONE', #102345, #52587, #83353 ) ;
#35404=VECTOR ( 'NONE', #29595, 1000.000000000000000 ) ;
#35405=ADVANCED_FACE ( 'NONE', ( #76953 ), #25922, .T. ) ;
#35406=VERTEX_POINT ( 'NONE', #65828 ) ;
#35408=CARTESIAN_POINT ( 'NONE',  ( 5.849999999999933031, 2.500000000000000000, -1.472243186433550122 ) ) ;
#35409=LINE ( 'NONE', #64848, #9283 ) ;
#35410=PLANE ( 'NONE',  #109270 ) ;
#35411=EDGE_CURVE ( 'NONE', #123035, #88198, #25635, .T. ) ;
#35412=DIRECTION ( 'NONE',  ( 0.000000000000000000, 0.000000000000000000, 1.000000000000000000 ) ) ;
#35413=ORIENTED_EDGE ( 'NONE', *, *, #29269, .T. ) ;
#35415=CARTESIAN_POINT ( 'NONE',  ( -3.350000000000028955, 2.500000000000000000, 2.165063509461097713 ) ) ;
#35417=ADVANCED_FACE ( 'NONE', ( #84180 ), #44514, .T. ) ;
#35418=EDGE_LOOP ( 'NONE', ( #58429, #87320 ) ) ;
#35419=DIRECTION ( 'NONE',  ( 0.000000000000000000, 1.000000000000000000, 0.000000000000000000 ) ) ;
#35420=ADVANCED_FACE ( 'NONE', ( #54715 ), #44922, .T. ) ;
#35421=ORIENTED_EDGE ( 'NONE', *, *, #116966, .F. ) ;
#35422=FACE_BOUND ( 'NONE', #123309, .T. ) ;
#35423=DIRECTION ( 'NONE',  ( -0.000000000000000000, 1.000000000000000000, -0.000000000000000000 ) ) ;
#35424=ADVANCED_FACE ( 'NONE', ( #6250 ), #46196, .T. ) ;
#35425=EDGE_CURVE ( 'NONE', #29584, #11046, #69546, .T. ) ;
#35426=ADVANCED_FACE ( 'NONE', ( #50096 ), #13397, .T. ) ;
#35427=EDGE_LOOP ( 'NONE', ( #120336, #51491, #121938, #63301 ) ) ;
#35428=DIRECTION ( 'NONE',  ( -0.000000000000000000, -1.000000000000000000, -0.000000000000000000 ) ) ;
#35429=CARTESIAN_POINT ( 'NONE',  ( -0.8500000000000382805, 2.500000000000000000, -1.372243186433550033 ) ) ;
#35430=ORIENTED_EDGE ( 'NONE', *, *, #59221, .F. ) ;
#35431=ORIENTED_EDGE ( 'NONE', *, *, #111788, .T. ) ;
#35433=AXIS2_PLACEMENT_3D ( 'NONE', #63019, #104232, #24386 ) ;
#35434=EDGE_CURVE ( 'NONE', #43040, #86788, #123925, .T. ) ;
#35435=ORIENTED_EDGE ( 'NONE', *, *, #33167, .T. ) ;
#35437=CARTESIAN_POINT ( 'NONE',  ( -2.700000000000029932, 2.500000000000000000, -4.676537180435977881 ) ) ;
#35438=DIRECTION ( 'NONE',  ( 0.000000000000000000, 0.000000000000000000, 1.000000000000000000 ) ) ;
#35439=LINE ( 'NONE', #103530, #9190 ) ;
#35440=DIRECTION ( 'NONE',  ( -0.000000000000000000, -1.000000000000000000, -0.000000000000000000 ) ) ;
#35441=CARTESIAN_POINT ( 'NONE',  ( 13.34999999999990017, 2.500000000000000000, 2.165063509461097713 ) ) ;
#35442=AXIS2_PLACEMENT_3D ( 'NONE', #10645, #11959, #30990 ) ;
#35443=VERTEX_POINT ( 'NONE', #40259 ) ;
#35444=VERTEX_POINT ( 'NONE', #19305 ) ;
#35445=CARTESIAN_POINT ( 'NONE',  ( -7.700000000000016165, 12.50000000000000000, -3.983716857408426293 ) ) ;
#35446=AXIS2_PLACEMENT_3D ( 'NONE', #101250, #39144, #31239 ) ;
#35448=CARTESIAN_POINT ( 'NONE',  ( 12.29999999999990479, 2.500000000000000000, 4.676537180435972552 ) ) ;
#35449=DIRECTION ( 'NONE',  ( -0.000000000000000000, 1.000000000000000000, -0.000000000000000000 ) ) ;
#35450=VECTOR ( 'NONE', #67620, 1000.000000000000000 ) ;
#35451=VERTEX_POINT ( 'NONE', #88028 ) ;
#35452=ORIENTED_EDGE ( 'NONE', *, *, #85886, .F. ) ;
#35453=FACE_BOUND ( 'NONE', #21898, .T. ) ;
#35454=ORIENTED_EDGE ( 'NONE', *, *, #54206, .T. ) ;
#35455=EDGE_CURVE ( 'NONE', #72066, #96049, #2639, .T. ) ;
#35456=DIRECTION ( 'NONE',  ( -0.000000000000000000, 1.000000000000000000, -0.000000000000000000 ) ) ;
#35457=CARTESIAN_POINT ( 'NONE',  ( 13.74999999999993072, 12.50000000000000000, -2.165063509461101710 ) ) ;
#35458=VERTEX_POINT ( 'NONE', #127985 ) ;
#35459=FACE_OUTER_BOUND ( 'NONE', #113070, .T. ) ;
#35460=VECTOR ( 'NONE', #37657, 1000.000000000000000 ) ;
#35461=DIRECTION ( 'NONE',  ( -0.000000000000000000, 1.000000000000000000, -0.000000000000000000 ) ) ;
#35462=DIRECTION ( 'NONE',  ( 0.000000000000000000, 0.000000000000000000, 1.000000000000000000 ) ) ;
#35463=FACE_OUTER_BOUND ( 'NONE', #68516, .T. ) ;
#35464=CARTESIAN_POINT ( 'NONE',  ( -0.8000000000000381251, 12.50000000000000000, 4.395220292106234439 ) ) ;
#35465=DIRECTION ( 'NONE',  ( -4.274815082592931898E-19, -0.9999939076577903929, -0.003490651415223739937 ) ) ;
#35468=DIRECTION ( 'NONE',  ( 0.000000000000000000, 0.000000000000000000, -1.000000000000000000 ) ) ;
#35469=ORIENTED_EDGE ( 'NONE', *, *, #70738, .T. ) ;
#35470=EDGE_CURVE ( 'NONE', #6533, #45263, #77963, .T. ) ;
#35471=EDGE_LOOP ( 'NONE', ( #72086, #126382, #94186, #30398 ) ) ;
#35472=DIRECTION ( 'NONE',  ( -0.000000000000000000, 1.000000000000000000, -0.000000000000000000 ) ) ;
#35473=VERTEX_POINT ( 'NONE', #38330 ) ;
#35474=CARTESIAN_POINT ( 'NONE',  ( -11.25000000000000000, 2.500000000000000000, -2.957883832488649833 ) ) ;
#35475=AXIS2_PLACEMENT_3D ( 'NONE', #107566, #57823, #80034 ) ;
#35476=VERTEX_POINT ( 'NONE', #69056 ) ;
#35477=ORIENTED_EDGE ( 'NONE', *, *, #73503, .T. ) ;
#35478=ORIENTED_EDGE ( 'NONE', *, *, #97301, .T. ) ;
#35479=DIRECTION ( 'NONE',  ( -4.274815082592931898E-19, -0.9999939076577903929, -0.003490651415223739937 ) ) ;
#35480=CIRCLE ( 'NONE', #89834, 0.06509327318403745899 ) ;
#35481=CONICAL_SURFACE ( 'NONE', #33431, 0.09999999999999999167, 0.003490658503988666988 ) ;
#35482=DIRECTION ( 'NONE',  ( 0.000000000000000000, 1.000000000000000000, 0.000000000000000000 ) ) ;
#35484=DIRECTION ( 'NONE',  ( 0.000000000000000000, -0.9999939076577903929, 0.003490651415223739937 ) ) ;
#35485=CARTESIAN_POINT ( 'NONE',  ( 3.149999999999942624, 12.50000000000000000, 6.776507416713035248 ) ) ;
#35486=CARTESIAN_POINT ( 'NONE',  ( 6.249999999999934275, 12.50000000000000000, -7.188010851410854052 ) ) ;
#35487=EDGE_CURVE ( 'NONE', #88829, #52488, #57024, .T. ) ;
#35488=EDGE_LOOP ( 'NONE', ( #29311, #122070 ) ) ;
#35489=VECTOR ( 'NONE', #123259, 1000.000000000000000 ) ;
#35490=VECTOR ( 'NONE', #83488, 1000.000000000000000 ) ;
#35491=DIRECTION ( 'NONE',  ( 0.000000000000000000, 0.000000000000000000, -1.000000000000000000 ) ) ;
#35492=CONICAL_SURFACE ( 'NONE', #6210, 0.1000000000000002554, 0.003490658503988666988 ) ;
#35493=VERTEX_POINT ( 'NONE', #57964 ) ;
#35494=ORIENTED_EDGE ( 'NONE', *, *, #6387, .F. ) ;
#35495=VERTEX_POINT ( 'NONE', #89354 ) ;
#35496=CARTESIAN_POINT ( 'NONE',  ( -7.100000000000017408, 2.500000000000000000, -0.6928203230275542523 ) ) ;
#35497=ORIENTED_EDGE ( 'NONE', *, *, #73031, .F. ) ;
#35498=VERTEX_POINT ( 'NONE', #28504 ) ;
#35499=EDGE_LOOP ( 'NONE', ( #79788, #67645, #78936, #46086 ) ) ;
#35500=AXIS2_PLACEMENT_3D ( 'NONE', #46682, #126535, #36871 ) ;
#35501=DIRECTION ( 'NONE',  ( -0.000000000000000000, -1.000000000000000000, -0.000000000000000000 ) ) ;
#35503=DIRECTION ( 'NONE',  ( 0.000000000000000000, 0.000000000000000000, 1.000000000000000000 ) ) ;
#35504=CARTESIAN_POINT ( 'NONE',  ( -9.800000000000004263, 12.50000000000000000, -0.3464101615137783474 ) ) ;
#35505=AXIS2_PLACEMENT_3D ( 'NONE', #66297, #125225, #115370 ) ;
#35506=DIRECTION ( 'NONE',  ( 0.000000000000000000, -0.000000000000000000, 1.000000000000000000 ) ) ;
#35507=FACE_OUTER_BOUND ( 'NONE', #58241, .T. ) ;
#35508=CARTESIAN_POINT ( 'NONE',  ( -6.900000000000019007, 2.500000000000000000, 0.2464101615137735679 ) ) ;
#35509=ORIENTED_EDGE ( 'NONE', *, *, #92391, .T. ) ;
#35510=CARTESIAN_POINT ( 'NONE',  ( -5.450000000000023270, 2.500000000000000000, -2.265063509461101798 ) ) ;
#35511=AXIS2_PLACEMENT_3D ( 'NONE', #83211, #84494, #124419 ) ;
#35512=EDGE_LOOP ( 'NONE', ( #112841, #19823 ) ) ;
#35513=CARTESIAN_POINT ( 'NONE',  ( 6.899999999999926636, 2.500000000000000000, -0.3464101615137782364 ) ) ;
#35514=EDGE_CURVE ( 'NONE', #24394, #114462, #11051, .T. ) ;
#35515=EDGE_LOOP ( 'NONE', ( #83371, #69777 ) ) ;
#35517=CIRCLE ( 'NONE', #54280, 0.06509327318403745899 ) ;
#35518=ORIENTED_EDGE ( 'NONE', *, *, #7640, .T. ) ;
#35520=ADVANCED_FACE ( 'NONE', ( #8838 ), #17293, .T. ) ;
#35521=LINE ( 'NONE', #95723, #36493 ) ;
#35522=CARTESIAN_POINT ( 'NONE',  ( 9.149999999999916866, 2.500000000000000000, -2.757883832488654097 ) ) ;
#35524=FACE_OUTER_BOUND ( 'NONE', #95406, .T. ) ;
#35525=ADVANCED_FACE ( 'NONE', ( #68410 ), #34062, .T. ) ;
#35526=CARTESIAN_POINT ( 'NONE',  ( 4.149999999999938183, 12.50000000000000000, 2.230156782645134950 ) ) ;
#35527=EDGE_CURVE ( 'NONE', #91704, #14107, #50784, .T. ) ;
#35528=ORIENTED_EDGE ( 'NONE', *, *, #2584, .F. ) ;
#35529=DIRECTION ( 'NONE',  ( 0.000000000000000000, -0.000000000000000000, 1.000000000000000000 ) ) ;
#35530=FACE_OUTER_BOUND ( 'NONE', #13230, .T. ) ;
#35531=EDGE_CURVE ( 'NONE', #39312, #91186, #59268, .T. ) ;
#35532=DIRECTION ( 'NONE',  ( -0.000000000000000000, 1.000000000000000000, -0.000000000000000000 ) ) ;
#35533=EDGE_CURVE ( 'NONE', #119152, #93088, #90467, .T. ) ;
#35534=ADVANCED_FACE ( 'NONE', ( #118806 ), #19971, .T. ) ;
#35535=PLANE ( 'NONE',  #101553 ) ;
#35536=DIRECTION ( 'NONE',  ( -4.274815082592931898E-19, -0.9999939076577903929, -0.003490651415223739937 ) ) ;
#35537=VERTEX_POINT ( 'NONE', #77577 ) ;
#35538=EDGE_LOOP ( 'NONE', ( #37605, #120729, #90476, #125857 ) ) ;
#35539=VECTOR ( 'NONE', #59494, 1000.000000000000000 ) ;
#35540=EDGE_CURVE ( 'NONE', #31716, #128537, #27846, .T. ) ;
#35541=VERTEX_POINT ( 'NONE', #108336 ) ;
#35542=EDGE_CURVE ( 'NONE', #102877, #36999, #86262, .T. ) ;
#35543=CARTESIAN_POINT ( 'NONE',  ( 9.149999999999915090, 2.500000000000000000, 6.495190528383297135 ) ) ;
#35544=CARTESIAN_POINT ( 'NONE',  ( 1.449999999999952216, 2.500000000000000000, -2.511473670974877948 ) ) ;
#35545=ADVANCED_FACE ( 'NONE', ( #97871 ), #61253, .T. ) ;
#35546=AXIS2_PLACEMENT_3D ( 'NONE', #28495, #67088, #116211 ) ;
#35548=DIRECTION ( 'NONE',  ( 0.000000000000000000, 0.000000000000000000, -1.000000000000000000 ) ) ;
#35549=DIRECTION ( 'NONE',  ( 0.000000000000000000, 0.000000000000000000, 1.000000000000000000 ) ) ;
#35550=DIRECTION ( 'NONE',  ( 0.000000000000000000, 0.000000000000000000, -1.000000000000000000 ) ) ;
#35551=DIRECTION ( 'NONE',  ( -4.274815082592931898E-19, -0.9999939076577903929, -0.003490651415223739937 ) ) ;
#35552=EDGE_LOOP ( 'NONE', ( #111031, #127674 ) ) ;
#35553=CIRCLE ( 'NONE', #50220, 0.09999999999999982514 ) ;
#35554=CONICAL_SURFACE ( 'NONE', #95895, 0.09999999999999982514, 0.003490658503988666988 ) ;
#35555=LINE ( 'NONE', #75456, #121251 ) ;
#35556=DIRECTION ( 'NONE',  ( 0.000000000000000000, 0.000000000000000000, 1.000000000000000000 ) ) ;
#35557=ORIENTED_EDGE ( 'NONE', *, *, #19214, .T. ) ;
#35558=CARTESIAN_POINT ( 'NONE',  ( -11.24999999999996447, 2.500000000000000000, -2.065063509461098068 ) ) ;
#35559=CARTESIAN_POINT ( 'NONE',  ( 7.099999999999926814, 2.500000000000000000, -0.5928203230275541635 ) ) ;
#35560=CARTESIAN_POINT ( 'NONE',  ( 3.949999999999942446, 2.500000000000000000, -2.611473670974877592 ) ) ;
#35562=DIRECTION ( 'NONE',  ( 0.000000000000000000, 0.000000000000000000, 1.000000000000000000 ) ) ;
#35563=EDGE_CURVE ( 'NONE', #33973, #129536, #103026, .T. ) ;
#35564=VERTEX_POINT ( 'NONE', #23175 ) ;
#35565=CARTESIAN_POINT ( 'NONE',  ( -1.450000000000035039, 12.50000000000000000, -2.511473670974877948 ) ) ;
#35566=LINE ( 'NONE', #76126, #11134 ) ;
#35567=EDGE_LOOP ( 'NONE', ( #119908, #123918 ) ) ;
#35568=AXIS2_PLACEMENT_3D ( 'NONE', #16298, #56237, #67988 ) ;
#35569=CARTESIAN_POINT ( 'NONE',  ( 4.349999999999938360, 2.500000000000000000, 1.718653347947321386 ) ) ;
#35570=CONICAL_SURFACE ( 'NONE', #16751, 0.09999999999999982514, 0.003490658503988666988 ) ;
#35571=EDGE_CURVE ( 'NONE', #9027, #82955, #65337, .T. ) ;
#35572=CARTESIAN_POINT ( 'NONE',  ( 12.49999999999990585, 2.500000000000000000, 3.637306695894644726 ) ) ;
#35573=EDGE_CURVE ( 'NONE', #108669, #71566, #4786, .T. ) ;
#35574=EDGE_LOOP ( 'NONE', ( #90453, #18028 ) ) ;
#35575=AXIS2_PLACEMENT_3D ( 'NONE', #38464, #117615, #79029 ) ;
#35576=CARTESIAN_POINT ( 'NONE',  ( -8.100000000000010303, 12.50000000000000000, 4.676537180435972552 ) ) ;
#35577=EDGE_CURVE ( 'NONE', #67278, #29034, #94684, .T. ) ;
#35578=ORIENTED_EDGE ( 'NONE', *, *, #91048, .T. ) ;
#35579=EDGE_CURVE ( 'NONE', #99488, #85816, #111394, .T. ) ;
#35581=PLANE ( 'NONE',  #46397 ) ;
#35582=CARTESIAN_POINT ( 'NONE',  ( -11.24999999999999822, 2.500000000000000000, 1.472243186433545459 ) ) ;
#35583=VERTEX_POINT ( 'NONE', #1600 ) ;
#35584=CIRCLE ( 'NONE', #79499, 0.1000000000000002554 ) ;
#35585=CARTESIAN_POINT ( 'NONE',  ( 2.949999999999946887, 12.50000000000000000, -2.165063509461101710 ) ) ;
#35586=DIRECTION ( 'NONE',  ( -4.274815082592931898E-19, -0.9999939076577903929, -0.003490651415223739937 ) ) ;
#35587=ORIENTED_EDGE ( 'NONE', *, *, #87568, .F. ) ;
#35588=ADVANCED_FACE ( 'NONE', ( #52637 ), #109261, .T. ) ;
#35589=VECTOR ( 'NONE', #97025, 1000.000000000000000 ) ;
#35590=DIRECTION ( 'NONE',  ( 0.000000000000000000, 1.000000000000000000, 0.000000000000000000 ) ) ;
#35591=DIRECTION ( 'NONE',  ( 0.000000000000000000, 0.000000000000000000, 1.000000000000000000 ) ) ;
#35592=CONICAL_SURFACE ( 'NONE', #16676, 0.09999999999999982514, 0.003490658503988666988 ) ;
#35593=CARTESIAN_POINT ( 'NONE',  ( 2.499999999999947153, 2.500000000000000000, 0.5928203230275495006 ) ) ;
#35594=CARTESIAN_POINT ( 'NONE',  ( 3.349999999999944578, 2.500000000000000000, -1.572243186433550211 ) ) ;
#35595=DIRECTION ( 'NONE',  ( -0.000000000000000000, -1.000000000000000000, -0.000000000000000000 ) ) ;
#35596=CARTESIAN_POINT ( 'NONE',  ( -4.600000000000024514, 12.50000000000000000, -0.7579135962115917113 ) ) ;
#35597=VECTOR ( 'NONE', #49741, 1000.000000000000000 ) ;
#35598=ORIENTED_EDGE ( 'NONE', *, *, #116245, .T. ) ;
#35599=ORIENTED_EDGE ( 'NONE', *, *, #83348, .T. ) ;
#35600=ORIENTED_EDGE ( 'NONE', *, *, #58314, .F. ) ;
#35601=VERTEX_POINT ( 'NONE', #111566 ) ;
#35602=AXIS2_PLACEMENT_3D ( 'NONE', #115895, #64219, #103510 ) ;
#35603=PLANE ( 'NONE',  #55786 ) ;
#35604=DIRECTION ( 'NONE',  ( 0.000000000000000000, 0.000000000000000000, 1.000000000000000000 ) ) ;
#35605=CARTESIAN_POINT ( 'NONE',  ( 10.59999999999991260, 12.50000000000000000, 0.3464101615137735735 ) ) ;
#35606=ORIENTED_EDGE ( 'NONE', *, *, #16753, .T. ) ;
#35607=FACE_BOUND ( 'NONE', #45316, .T. ) ;
#35608=ADVANCED_FACE ( 'NONE', ( #12070 ), #2737, .T. ) ;
#35609=CARTESIAN_POINT ( 'NONE',  ( -1.250000000000001110, 2.500000000000000000, -2.065063509461102065 ) ) ;
#35610=LINE ( 'NONE', #66969, #89811 ) ;
#35611=DIRECTION ( 'NONE',  ( 0.000000000000000000, 0.000000000000000000, -1.000000000000000000 ) ) ;
#35612=CARTESIAN_POINT ( 'NONE',  ( -3.470457856696441969E-14, 12.50000000000000000, -0.7579135962115893799 ) ) ;
#35613=PLANE ( 'NONE',  #80632 ) ;
#35614=DIRECTION ( 'NONE',  ( -4.274815082592931898E-19, -0.9999939076577903929, -0.003490651415223739937 ) ) ;
#35615=FACE_OUTER_BOUND ( 'NONE', #122255, .T. ) ;
#35616=CARTESIAN_POINT ( 'NONE',  ( 12.69999999999990159, 12.50000000000000000, -3.983716857408426293 ) ) ;
#35617=DIRECTION ( 'NONE',  ( 0.000000000000000000, 1.000000000000000000, 0.000000000000000000 ) ) ;
#35618=CARTESIAN_POINT ( 'NONE',  ( 0.8499999999999553468, 12.50000000000000000, -2.792790559304616504 ) ) ;
#35619=EDGE_LOOP ( 'NONE', ( #60085, #90611, #96906, #52151 ) ) ;
#35620=ORIENTED_EDGE ( 'NONE', *, *, #107356, .T. ) ;
#35621=EDGE_CURVE ( 'NONE', #118275, #79663, #8997, .T. ) ;
#35622=ORIENTED_EDGE ( 'NONE', *, *, #23441, .T. ) ;
#35623=EDGE_LOOP ( 'NONE', ( #64684, #120445 ) ) ;
#35624=DIRECTION ( 'NONE',  ( 0.000000000000000000, 1.000000000000000000, 0.000000000000000000 ) ) ;
#35625=ORIENTED_EDGE ( 'NONE', *, *, #113727, .F. ) ;
#35626=AXIS2_PLACEMENT_3D ( 'NONE', #70419, #62544, #110341 ) ;
#35627=DIRECTION ( 'NONE',  ( 0.000000000000000000, 0.000000000000000000, 1.000000000000000000 ) ) ;
#35628=CONICAL_SURFACE ( 'NONE', #106702, 0.09999999999999982514, 0.003490658503988666988 ) ;
#35629=EDGE_LOOP ( 'NONE', ( #24244, #75009 ) ) ;
#35630=ORIENTED_EDGE ( 'NONE', *, *, #27680, .T. ) ;
#35631=DIRECTION ( 'NONE',  ( -0.000000000000000000, 1.000000000000000000, -0.000000000000000000 ) ) ;
#35632=AXIS2_PLACEMENT_3D ( 'NONE', #119390, #31672, #70951 ) ;
#35633=AXIS2_PLACEMENT_3D ( 'NONE', #123942, #34305, #82763 ) ;
#35634=CARTESIAN_POINT ( 'NONE',  ( 12.69999999999990337, 2.500000000000000000, 4.083716857408420609 ) ) ;
#35635=DIRECTION ( 'NONE',  ( 0.000000000000000000, -0.000000000000000000, 1.000000000000000000 ) ) ;
#35636=CARTESIAN_POINT ( 'NONE',  ( -3.100000000000028955, 12.50000000000000000, 4.048810130592458201 ) ) ;
#35637=LINE ( 'NONE', #16614, #45627 ) ;
#35639=ORIENTED_EDGE ( 'NONE', *, *, #74408, .T. ) ;
#35640=VERTEX_POINT ( 'NONE', #21913 ) ;
#35641=EDGE_LOOP ( 'NONE', ( #27184, #99266, #44708, #95953 ) ) ;
#35642=CARTESIAN_POINT ( 'NONE',  ( 2.699999999999944666, 12.50000000000000000, 4.611443907251934426 ) ) ;
#35643=ORIENTED_EDGE ( 'NONE', *, *, #37293, .F. ) ;
#35644=FACE_OUTER_BOUND ( 'NONE', #107158, .T. ) ;
#35645=ORIENTED_EDGE ( 'NONE', *, *, #45383, .T. ) ;
#35647=LINE ( 'NONE', #84738, #102815 ) ;
#35648=DIRECTION ( 'NONE',  ( 0.000000000000000000, -0.9999939076577903929, 0.003490651415223739937 ) ) ;
#35649=FACE_OUTER_BOUND ( 'NONE', #108948, .T. ) ;
#35651=FACE_OUTER_BOUND ( 'NONE', #106784, .T. ) ;
#35652=LINE ( 'NONE', #115467, #30929 ) ;
#35653=ORIENTED_EDGE ( 'NONE', *, *, #93165, .F. ) ;
#35654=CARTESIAN_POINT ( 'NONE',  ( 1.249999999999952482, 2.500000000000000000, -5.702370205355749455 ) ) ;
#35655=AXIS2_PLACEMENT_3D ( 'NONE', #70765, #32151, #51775 ) ;
#35656=CONICAL_SURFACE ( 'NONE', #56563, 0.1000000000000002554, 0.003490658503988666988 ) ;
#35657=EDGE_LOOP ( 'NONE', ( #120539, #7041, #127706, #90872 ) ) ;
#35658=CARTESIAN_POINT ( 'NONE',  ( -3.150000000000030109, 2.500000000000000000, 1.818653347947321475 ) ) ;
#35660=EDGE_LOOP ( 'NONE', ( #67931, #15472, #92931, #40023 ) ) ;
#35661=DIRECTION ( 'NONE',  ( 0.000000000000000000, 0.000000000000000000, 1.000000000000000000 ) ) ;
#35662=CARTESIAN_POINT ( 'NONE',  ( -3.300000000000027800, 12.50000000000000000, -4.330127018922201643 ) ) ;
#35663=ORIENTED_EDGE ( 'NONE', *, *, #7743, .T. ) ;
#35664=DIRECTION ( 'NONE',  ( -0.000000000000000000, 1.000000000000000000, -0.000000000000000000 ) ) ;
#35665=DIRECTION ( 'NONE',  ( 0.000000000000000000, 1.000000000000000000, 0.000000000000000000 ) ) ;
#35666=ORIENTED_EDGE ( 'NONE', *, *, #59804, .F. ) ;
#35667=AXIS2_PLACEMENT_3D ( 'NONE', #79653, #11551, #121494 ) ;
#35668=EDGE_CURVE ( 'NONE', #92847, #47032, #63395, .T. ) ;
#35669=DIRECTION ( 'NONE',  ( 0.000000000000000000, 0.000000000000000000, 1.000000000000000000 ) ) ;
#35670=CARTESIAN_POINT ( 'NONE',  ( -11.44999999999999751, 2.500000000000000000, -2.511473670974873951 ) ) ;
#35671=ORIENTED_EDGE ( 'NONE', *, *, #16173, .F. ) ;
#35672=EDGE_CURVE ( 'NONE', #10174, #96773, #33028, .T. ) ;
#35673=EDGE_CURVE ( 'NONE', #34505, #39201, #110276, .T. ) ;
#35674=VERTEX_POINT ( 'NONE', #92571 ) ;
#35675=DIRECTION ( 'NONE',  ( -0.000000000000000000, -1.000000000000000000, -0.000000000000000000 ) ) ;
#35676=DIRECTION ( 'NONE',  ( -0.000000000000000000, 1.000000000000000000, -0.000000000000000000 ) ) ;
#35677=ADVANCED_FACE ( 'NONE', ( #112216 ), #119825, .T. ) ;
#35679=EDGE_CURVE ( 'NONE', #5496, #63429, #117746, .T. ) ;
#35680=DIRECTION ( 'NONE',  ( 0.000000000000000000, 0.000000000000000000, -1.000000000000000000 ) ) ;
#35681=CIRCLE ( 'NONE', #98347, 0.1000000000000002554 ) ;
#35682=CIRCLE ( 'NONE', #29333, 0.1000000000000002554 ) ;
#35683=CARTESIAN_POINT ( 'NONE',  ( -6.650000000000018119, 2.500000000000000000, -6.495190528383302464 ) ) ;
#35684=CARTESIAN_POINT ( 'NONE',  ( -11.24999999999999822, 2.500000000000000000, 5.802370205355744659 ) ) ;
#35685=EDGE_CURVE ( 'NONE', #123334, #113423, #121875, .T. ) ;
#35686=EDGE_CURVE ( 'NONE', #96252, #85559, #52930, .T. ) ;
#35687=EDGE_CURVE ( 'NONE', #115043, #43214, #46670, .T. ) ;
#35688=CONICAL_SURFACE ( 'NONE', #79597, 0.1000000000000002554, 0.003490658503988666988 ) ;
#35689=VERTEX_POINT ( 'NONE', #55232 ) ;
#35690=EDGE_CURVE ( 'NONE', #97645, #72180, #4880, .T. ) ;
#35691=LINE ( 'NONE', #76261, #38092 ) ;
#35692=ADVANCED_FACE ( 'NONE', ( #84679 ), #69649, .T. ) ;
#35693=EDGE_LOOP ( 'NONE', ( #102139, #22596 ) ) ;
#35694=AXIS2_PLACEMENT_3D ( 'NONE', #86104, #102695, #75023 ) ;
#35695=FACE_OUTER_BOUND ( 'NONE', #30823, .T. ) ;
#35696=FACE_OUTER_BOUND ( 'NONE', #21119, .T. ) ;
#35697=CARTESIAN_POINT ( 'NONE',  ( -0.4000000000000331624, 2.500000000000000000, -0.1000000000000000056 ) ) ;
#35699=EDGE_LOOP ( 'NONE', ( #47894, #118634, #118772, #14697 ) ) ;
#35700=CARTESIAN_POINT ( 'NONE',  ( -10.85000000000000142, 12.50000000000000000, -6.430097255199260786 ) ) ;
#35701=CARTESIAN_POINT ( 'NONE',  ( -8.350000000000013856, 2.500000000000000000, 2.065063509461097624 ) ) ;
#35702=VERTEX_POINT ( 'NONE', #125253 ) ;
#35703=DIRECTION ( 'NONE',  ( -0.000000000000000000, -1.000000000000000000, -0.000000000000000000 ) ) ;
#35704=ORIENTED_EDGE ( 'NONE', *, *, #13465, .F. ) ;
#35705=ORIENTED_EDGE ( 'NONE', *, *, #37731, .F. ) ;
#35706=DIRECTION ( 'NONE',  ( 0.000000000000000000, 1.000000000000000000, 0.000000000000000000 ) ) ;
#35707=AXIS2_PLACEMENT_3D ( 'NONE', #13739, #44502, #101502 ) ;
#35708=AXIS2_PLACEMENT_3D ( 'NONE', #77511, #38249, #19220 ) ;
#35709=VECTOR ( 'NONE', #60615, 1000.000000000000000 ) ;
#35710=EDGE_LOOP ( 'NONE', ( #20418, #83617 ) ) ;
#35711=CARTESIAN_POINT ( 'NONE',  ( 6.899999999999926636, 12.50000000000000000, 0.3464101615137736845 ) ) ;
#35712=CARTESIAN_POINT ( 'NONE',  ( -8.350000000000013856, 2.500000000000000000, -5.802370205355744659 ) ) ;
#35713=CARTESIAN_POINT ( 'NONE',  ( -6.250000000000019540, 2.500000000000000000, -7.188010851410854052 ) ) ;
#35714=ORIENTED_EDGE ( 'NONE', *, *, #6378, .F. ) ;
#35715=FACE_BOUND ( 'NONE', #83113, .T. ) ;
#35716=DIRECTION ( 'NONE',  ( -0.000000000000000000, 1.000000000000000000, -0.000000000000000000 ) ) ;
#35717=ORIENTED_EDGE ( 'NONE', *, *, #88568, .T. ) ;
#35718=CIRCLE ( 'NONE', #102610, 0.06509327318403745899 ) ;
#35719=DIRECTION ( 'NONE',  ( 0.000000000000000000, 1.000000000000000000, 0.000000000000000000 ) ) ;
#35720=DIRECTION ( 'NONE',  ( -0.000000000000000000, -1.000000000000000000, -0.000000000000000000 ) ) ;
#35721=EDGE_LOOP ( 'NONE', ( #47780, #5901, #33395, #20332 ) ) ;
#35722=EDGE_CURVE ( 'NONE', #112193, #62955, #11149, .T. ) ;
#35723=ORIENTED_EDGE ( 'NONE', *, *, #72061, .F. ) ;
#35724=ADVANCED_FACE ( 'NONE', ( #6103 ), #95791, .T. ) ;
#35725=ORIENTED_EDGE ( 'NONE', *, *, #85265, .F. ) ;
#35726=PLANE ( 'NONE',  #25277 ) ;
#35727=FACE_OUTER_BOUND ( 'NONE', #100975, .T. ) ;
#35728=DIRECTION ( 'NONE',  ( 0.000000000000000000, 1.000000000000000000, 0.000000000000000000 ) ) ;
#35729=FACE_BOUND ( 'NONE', #55784, .T. ) ;
#35730=VERTEX_POINT ( 'NONE', #54559 ) ;
#35732=EDGE_CURVE ( 'NONE', #98489, #79642, #6729, .T. ) ;
#35733=DIRECTION ( 'NONE',  ( 0.000000000000000000, 1.000000000000000000, 0.000000000000000000 ) ) ;
#35734=CARTESIAN_POINT ( 'NONE',  ( 7.049999999999928768, 2.500000000000000000, 6.595190528383296780 ) ) ;
#35735=EDGE_CURVE ( 'NONE', #31758, #15286, #75906, .T. ) ;
#35736=AXIS2_PLACEMENT_3D ( 'NONE', #15635, #4511, #123041 ) ;
#35737=DIRECTION ( 'NONE',  ( 0.000000000000000000, -0.9999939076577903929, 0.003490651415223739937 ) ) ;
#35738=EDGE_CURVE ( 'NONE', #781, #63941, #36240, .T. ) ;
#35739=CARTESIAN_POINT ( 'NONE',  ( -0.4000000000000339950, 2.500000000000000000, 0.6928203230275518099 ) ) ;
#35740=LINE ( 'NONE', #95305, #71917 ) ;
#35741=CARTESIAN_POINT ( 'NONE',  ( 4.149999999999938183, 2.500000000000000000, 7.088010851410848190 ) ) ;
#35742=CARTESIAN_POINT ( 'NONE',  ( 10.44999999999991402, 2.500000000000000000, -2.165063509461101710 ) ) ;
#35743=CIRCLE ( 'NONE', #108883, 0.06509327318403745899 ) ;
#35744=CIRCLE ( 'NONE', #50401, 0.1000000000000000472 ) ;
#35745=DIRECTION ( 'NONE',  ( 0.000000000000000000, 0.000000000000000000, 1.000000000000000000 ) ) ;
#35746=ORIENTED_EDGE ( 'NONE', *, *, #9099, .T. ) ;
#35747=ORIENTED_EDGE ( 'NONE', *, *, #80782, .T. ) ;
#35748=ORIENTED_EDGE ( 'NONE', *, *, #74097, .T. ) ;
#35749=ORIENTED_EDGE ( 'NONE', *, *, #72716, .F. ) ;
#35750=ORIENTED_EDGE ( 'NONE', *, *, #40994, .F. ) ;
#35752=DIRECTION ( 'NONE',  ( 0.000000000000000000, 1.000000000000000000, 0.000000000000000000 ) ) ;
#35753=ORIENTED_EDGE ( 'NONE', *, *, #53265, .F. ) ;
#35754=FACE_BOUND ( 'NONE', #53126, .T. ) ;
#35755=CIRCLE ( 'NONE', #62935, 0.1000000000000000472 ) ;
#35756=DIRECTION ( 'NONE',  ( 0.000000000000000000, 1.000000000000000000, 0.000000000000000000 ) ) ;
#35757=CIRCLE ( 'NONE', #96372, 0.1000000000000002554 ) ;
#35758=DIRECTION ( 'NONE',  ( 0.000000000000000000, 0.000000000000000000, 1.000000000000000000 ) ) ;
#35759=ORIENTED_EDGE ( 'NONE', *, *, #111623, .F. ) ;
#35760=LINE ( 'NONE', #106426, #5610 ) ;
#35761=FACE_OUTER_BOUND ( 'NONE', #56875, .T. ) ;
#35762=CARTESIAN_POINT ( 'NONE',  ( -15.19999999999998330, 2.500000000000000000, 0.4464101615137758272 ) ) ;
#35763=ORIENTED_EDGE ( 'NONE', *, *, #60515, .T. ) ;
#35764=LINE ( 'NONE', #35139, #57713 ) ;
#35767=ORIENTED_EDGE ( 'NONE', *, *, #26864, .T. ) ;
#35768=AXIS2_PLACEMENT_3D ( 'NONE', #120250, #82259, #12832 ) ;
#35769=ORIENTED_EDGE ( 'NONE', *, *, #121234, .F. ) ;
#35770=ORIENTED_EDGE ( 'NONE', *, *, #119416, .F. ) ;
#35771=CARTESIAN_POINT ( 'NONE',  ( 1.849999999999949685, 2.500000000000000000, -2.611473670974877592 ) ) ;
#35772=DIRECTION ( 'NONE',  ( -0.000000000000000000, -1.000000000000000000, -0.000000000000000000 ) ) ;
#35773=DIRECTION ( 'NONE',  ( -0.000000000000000000, -1.000000000000000000, -0.000000000000000000 ) ) ;
#35774=ORIENTED_EDGE ( 'NONE', *, *, #90865, .T. ) ;
#35775=CARTESIAN_POINT ( 'NONE',  ( 15.23091471310319278, 2.499999999999935163, -7.179421168902959671 ) ) ;
#35776=VECTOR ( 'NONE', #106393, 1000.000000000000000 ) ;
#35777=DIRECTION ( 'NONE',  ( 0.000000000000000000, 0.000000000000000000, -1.000000000000000000 ) ) ;
#35778=DIRECTION ( 'NONE',  ( 0.000000000000000000, 1.000000000000000000, 0.000000000000000000 ) ) ;
#35779=AXIS2_PLACEMENT_3D ( 'NONE', #13357, #2913, #53307 ) ;
#35780=AXIS2_PLACEMENT_3D ( 'NONE', #64620, #23399, #73792 ) ;
#35782=CARTESIAN_POINT ( 'NONE',  ( 1.649999999999951505, 2.500000000000000000, 1.572243186433545548 ) ) ;
#35783=ADVANCED_FACE ( 'NONE', ( #93860 ), #25728, .T. ) ;
#35784=CARTESIAN_POINT ( 'NONE',  ( 2.499999999999947153, 2.500000000000000000, 3.637306695894644726 ) ) ;
#35785=EDGE_CURVE ( 'NONE', #47693, #75963, #98891, .T. ) ;
#35786=ORIENTED_EDGE ( 'NONE', *, *, #86285, .F. ) ;
#35787=DIRECTION ( 'NONE',  ( 0.000000000000000000, 0.000000000000000000, -1.000000000000000000 ) ) ;
#35788=ORIENTED_EDGE ( 'NONE', *, *, #26506, .T. ) ;
#35789=ORIENTED_EDGE ( 'NONE', *, *, #10663, .T. ) ;
#35790=DIRECTION ( 'NONE',  ( 0.000000000000000000, -0.000000000000000000, 1.000000000000000000 ) ) ;
#35791=DIRECTION ( 'NONE',  ( 0.000000000000000000, 1.000000000000000000, 0.000000000000000000 ) ) ;
#35792=DIRECTION ( 'NONE',  ( -0.000000000000000000, 1.000000000000000000, -0.000000000000000000 ) ) ;
#35793=ADVANCED_FACE ( 'NONE', ( #124613 ), #90573, .T. ) ;
#35794=ORIENTED_EDGE ( 'NONE', *, *, #6090, .T. ) ;
#35795=ORIENTED_EDGE ( 'NONE', *, *, #58208, .T. ) ;
#35796=DIRECTION ( 'NONE',  ( -0.000000000000000000, 1.000000000000000000, -0.000000000000000000 ) ) ;
#35797=CARTESIAN_POINT ( 'NONE',  ( 81.97074731400692826, 3.937872643741660017, -6.123955218199263584 ) ) ;
#35798=CIRCLE ( 'NONE', #33741, 0.1000000000000002554 ) ;
#35799=DIRECTION ( 'NONE',  ( -0.000000000000000000, -1.000000000000000000, -0.000000000000000000 ) ) ;
#35800=ORIENTED_EDGE ( 'NONE', *, *, #60264, .T. ) ;
#35801=ORIENTED_EDGE ( 'NONE', *, *, #73114, .T. ) ;
#35802=AXIS2_PLACEMENT_3D ( 'NONE', #43747, #41324, #89755 ) ;
#35803=CIRCLE ( 'NONE', #273, 0.1000000000000002554 ) ;
#35804=FACE_OUTER_BOUND ( 'NONE', #94569, .T. ) ;
#35805=ORIENTED_EDGE ( 'NONE', *, *, #103403, .T. ) ;
#35806=DIRECTION ( 'NONE',  ( 0.000000000000000000, 0.000000000000000000, -1.000000000000000000 ) ) ;
#35807=AXIS2_PLACEMENT_3D ( 'NONE', #86398, #116508, #10427 ) ;
#35808=DIRECTION ( 'NONE',  ( 0.000000000000000000, -0.000000000000000000, 1.000000000000000000 ) ) ;
#35809=ORIENTED_EDGE ( 'NONE', *, *, #51214, .T. ) ;
#35810=DIRECTION ( 'NONE',  ( -0.000000000000000000, -1.000000000000000000, -0.000000000000000000 ) ) ;
#35811=CARTESIAN_POINT ( 'NONE',  ( 10.84999999999990905, 12.50000000000000000, 1.407149913249508000 ) ) ;
#35812=DIRECTION ( 'NONE',  ( -0.000000000000000000, 1.000000000000000000, -0.000000000000000000 ) ) ;
#35813=AXIS2_PLACEMENT_3D ( 'NONE', #124670, #55913, #64445 ) ;
#35814=LINE ( 'NONE', #87474, #66762 ) ;
#35815=EDGE_LOOP ( 'NONE', ( #68420, #102635, #38689, #1276 ) ) ;
#35816=EDGE_CURVE ( 'NONE', #89205, #7349, #115604, .T. ) ;
#35817=FACE_OUTER_BOUND ( 'NONE', #124927, .T. ) ;
#35818=LINE ( 'NONE', #75730, #10226 ) ;
#35819=EDGE_LOOP ( 'NONE', ( #6361, #86541 ) ) ;
#35820=EDGE_LOOP ( 'NONE', ( #12727, #76975 ) ) ;
#35821=ADVANCED_FACE ( 'NONE', ( #15923 ), #53938, .T. ) ;
#35822=EDGE_CURVE ( 'NONE', #98931, #22721, #107300, .T. ) ;
#35824=FACE_OUTER_BOUND ( 'NONE', #24729, .T. ) ;
#35825=CARTESIAN_POINT ( 'NONE',  ( -12.49999999999995914, 12.50000000000000000, -4.330127018922198978 ) ) ;
#35826=EDGE_CURVE ( 'NONE', #127250, #107780, #115395, .T. ) ;
#35827=DIRECTION ( 'NONE',  ( 0.000000000000000000, 0.000000000000000000, 1.000000000000000000 ) ) ;
#35828=EDGE_CURVE ( 'NONE', #74205, #65138, #44609, .T. ) ;
#35829=CARTESIAN_POINT ( 'NONE',  ( -6.900000000000019007, 12.50000000000000000, 0.3464101615137735735 ) ) ;
#35830=CARTESIAN_POINT ( 'NONE',  ( 3.149999999999944400, 2.500000000000000000, 2.511473670974873507 ) ) ;
#35832=CARTESIAN_POINT ( 'NONE',  ( -4.150000000000025224, 12.50000000000000000, 7.188010851410848723 ) ) ;
#35833=DIRECTION ( 'NONE',  ( 0.000000000000000000, 0.000000000000000000, 1.000000000000000000 ) ) ;
#35834=EDGE_CURVE ( 'NONE', #123777, #62546, #65678, .T. ) ;
#35835=ADVANCED_FACE ( 'NONE', ( #129149 ), #71805, .T. ) ;
#35836=CARTESIAN_POINT ( 'NONE',  ( -7.900000000000011013, 12.50000000000000000, 3.637306695894644726 ) ) ;
#35837=CONICAL_SURFACE ( 'NONE', #12818, 0.1000000000000002554, 0.003490658503988666988 ) ;
#35838=VERTEX_POINT ( 'NONE', #59760 ) ;
#35839=AXIS2_PLACEMENT_3D ( 'NONE', #121952, #93142, #43411 ) ;
#35840=EDGE_CURVE ( 'NONE', #46113, #23974, #116709, .T. ) ;
#35841=ORIENTED_EDGE ( 'NONE', *, *, #77357, .F. ) ;
#35842=ORIENTED_EDGE ( 'NONE', *, *, #28433, .T. ) ;
#35843=EDGE_CURVE ( 'NONE', #89842, #27226, #126548, .T. ) ;
#35844=CARTESIAN_POINT ( 'NONE',  ( 5.649999999999932854, 12.50000000000000000, 2.446380397790835826 ) ) ;
#35845=DIRECTION ( 'NONE',  ( 0.000000000000000000, 0.000000000000000000, -1.000000000000000000 ) ) ;
#35846=DIRECTION ( 'NONE',  ( 0.000000000000000000, 0.000000000000000000, -1.000000000000000000 ) ) ;
#35847=CIRCLE ( 'NONE', #117379, 0.1000000000000000472 ) ;
#35848=EDGE_CURVE ( 'NONE', #122177, #81286, #128253, .T. ) ;
#35849=CIRCLE ( 'NONE', #6554, 0.09999999999999982514 ) ;
#35850=ORIENTED_EDGE ( 'NONE', *, *, #98379, .F. ) ;
#35851=LINE ( 'NONE', #6352, #123994 ) ;
#35852=CARTESIAN_POINT ( 'NONE',  ( -4.800000000000024691, 2.500000000000000000, 4.576537180435972019 ) ) ;
#35853=CARTESIAN_POINT ( 'NONE',  ( 1.699999999999951994, 2.500000000000000000, -4.230127018922201998 ) ) ;
#35854=ORIENTED_EDGE ( 'NONE', *, *, #17031, .T. ) ;
#35855=FACE_OUTER_BOUND ( 'NONE', #52202, .T. ) ;
#35856=CIRCLE ( 'NONE', #90121, 0.1000000000000002554 ) ;
#35857=ORIENTED_EDGE ( 'NONE', *, *, #84329, .T. ) ;
#35858=DIRECTION ( 'NONE',  ( 0.000000000000000000, 0.000000000000000000, -1.000000000000000000 ) ) ;
#35859=AXIS2_PLACEMENT_3D ( 'NONE', #78241, #18006, #117467 ) ;
#35860=ORIENTED_EDGE ( 'NONE', *, *, #13667, .F. ) ;
#35861=VERTEX_POINT ( 'NONE', #109481 ) ;
#35862=CONICAL_SURFACE ( 'NONE', #79776, 0.1000000000000000056, 0.003490658503988666988 ) ;
#35863=ORIENTED_EDGE ( 'NONE', *, *, #29892, .T. ) ;
#35864=CARTESIAN_POINT ( 'NONE',  ( 3.549999999999940314, 2.500000000000000000, 6.841600689897072485 ) ) ;
#35865=AXIS2_PLACEMENT_3D ( 'NONE', #13336, #10743, #112850 ) ;
#35866=PLANE ( 'NONE',  #44608 ) ;
#35868=CARTESIAN_POINT ( 'NONE',  ( -5.850000000000018296, 2.500000000000000000, 5.802370205355744659 ) ) ;
#35869=ORIENTED_EDGE ( 'NONE', *, *, #45605, .T. ) ;
#35870=AXIS2_PLACEMENT_3D ( 'NONE', #34318, #74224, #15925 ) ;
#35871=AXIS2_PLACEMENT_3D ( 'NONE', #73633, #4886, #62553 ) ;
#35872=DIRECTION ( 'NONE',  ( 0.000000000000000000, 0.000000000000000000, 1.000000000000000000 ) ) ;
#35873=ORIENTED_EDGE ( 'NONE', *, *, #118587, .T. ) ;
#35874=CARTESIAN_POINT ( 'NONE',  ( 76.40063402985219909, -3.742348971402477353, -5.987205606701297533 ) ) ;
#35875=CARTESIAN_POINT ( 'NONE',  ( 13.92826132181480681, -2.499999999999999112, -6.790916467786979993 ) ) ;
#35876=DIRECTION ( 'NONE',  ( -0.000000000000000000, 1.000000000000000000, -0.000000000000000000 ) ) ;
#35877=CARTESIAN_POINT ( 'NONE',  ( 16.72050902517240800, -2.552201582239431943, 5.918448581780632267 ) ) ;
#35878=ORIENTED_EDGE ( 'NONE', *, *, #26972, .F. ) ;
#35879=ADVANCED_FACE ( 'NONE', ( #28997 ), #21723, .T. ) ;
#35880=EDGE_LOOP ( 'NONE', ( #114337, #25593 ) ) ;
#35881=EDGE_CURVE ( 'NONE', #103364, #4955, #128147, .T. ) ;
#35882=ORIENTED_EDGE ( 'NONE', *, *, #4058, .T. ) ;
#35883=CARTESIAN_POINT ( 'NONE',  ( -12.09999999999999432, 12.50000000000000000, 5.022947341949748790 ) ) ;
#35884=DIRECTION ( 'NONE',  ( -0.000000000000000000, -1.000000000000000000, -0.000000000000000000 ) ) ;
#35885=DIRECTION ( 'NONE',  ( 0.000000000000000000, 0.000000000000000000, 1.000000000000000000 ) ) ;
#35886=FACE_BOUND ( 'NONE', #84810, .T. ) ;
#35887=CARTESIAN_POINT ( 'NONE',  ( -4.600000000000025402, 2.500000000000000000, 4.330127018922196314 ) ) ;
#35888=DIRECTION ( 'NONE',  ( -0.000000000000000000, 1.000000000000000000, -0.000000000000000000 ) ) ;
#35889=CARTESIAN_POINT ( 'NONE',  ( -8.350000000000013856, 12.50000000000000000, 2.165063509461097713 ) ) ;
#35890=CARTESIAN_POINT ( 'NONE',  ( -4.999999999999990230, 2.500000000000000000, -4.230127018922201998 ) ) ;
#35891=AXIS2_PLACEMENT_3D ( 'NONE', #93524, #113157, #23487 ) ;
#35893=AXIS2_PLACEMENT_3D ( 'NONE', #106793, #38745, #17099 ) ;
#35894=DIRECTION ( 'NONE',  ( -4.274815082592931898E-19, -0.9999939076577903929, -0.003490651415223739937 ) ) ;
#35895=DIRECTION ( 'NONE',  ( 0.000000000000000000, -0.000000000000000000, 1.000000000000000000 ) ) ;
#35896=AXIS2_PLACEMENT_3D ( 'NONE', #116353, #35876, #95442 ) ;
#35897=CARTESIAN_POINT ( 'NONE',  ( 8.549999999999922551, 12.50000000000000000, 2.576566944158910744 ) ) ;
#35898=CONICAL_SURFACE ( 'NONE', #19143, 0.1000000000000002554, 0.003490658503988666988 ) ;
#35899=VERTEX_POINT ( 'NONE', #99669 ) ;
#35900=ORIENTED_EDGE ( 'NONE', *, *, #45438, .T. ) ;
#35901=ORIENTED_EDGE ( 'NONE', *, *, #96496, .F. ) ;
#35902=ORIENTED_EDGE ( 'NONE', *, *, #20594, .F. ) ;
#35903=CONICAL_SURFACE ( 'NONE', #29640, 0.09999999999999999167, 0.003490658503988666988 ) ;
#35904=CARTESIAN_POINT ( 'NONE',  ( -8.750000000000012434, 2.500000000000000000, -5.902370205355745192 ) ) ;
#35905=FACE_BOUND ( 'NONE', #58546, .T. ) ;
#35906=DIRECTION ( 'NONE',  ( 0.000000000000000000, 0.000000000000000000, -1.000000000000000000 ) ) ;
#35907=AXIS2_PLACEMENT_3D ( 'NONE', #78271, #19981, #86769 ) ;
#35908=ORIENTED_EDGE ( 'NONE', *, *, #54603, .F. ) ;
#35909=DIRECTION ( 'NONE',  ( -0.000000000000000000, -1.000000000000000000, -0.000000000000000000 ) ) ;
#35910=DIRECTION ( 'NONE',  ( 0.000000000000000000, 0.000000000000000000, -1.000000000000000000 ) ) ;
#35911=ORIENTED_EDGE ( 'NONE', *, *, #67128, .T. ) ;
#35913=CARTESIAN_POINT ( 'NONE',  ( 0.6499999999999566125, 2.500000000000000000, -6.148780366869526226 ) ) ;
#35914=EDGE_CURVE ( 'NONE', #32951, #18013, #107390, .T. ) ;
#35915=EDGE_LOOP ( 'NONE', ( #77421, #35144, #40405, #98151 ) ) ;
#35916=DIRECTION ( 'NONE',  ( 0.000000000000000000, 1.000000000000000000, 0.000000000000000000 ) ) ;
#35917=DIRECTION ( 'NONE',  ( -4.274815082592931898E-19, -0.9999939076577903929, -0.003490651415223739937 ) ) ;
#35918=CONICAL_SURFACE ( 'NONE', #75714, 0.1000000000000000472, 0.003490658503988666988 ) ;
#35919=EDGE_CURVE ( 'NONE', #124332, #59408, #9990, .T. ) ;
#35920=CIRCLE ( 'NONE', #109056, 0.06509327318403745899 ) ;
#35921=ORIENTED_EDGE ( 'NONE', *, *, #76206, .F. ) ;
#35922=CARTESIAN_POINT ( 'NONE',  ( -7.700000000000016165, 2.500000000000000000, 0.2464101615137735679 ) ) ;
#35923=FACE_OUTER_BOUND ( 'NONE', #52264, .T. ) ;
#35924=VERTEX_POINT ( 'NONE', #7392 ) ;
#35925=CARTESIAN_POINT ( 'NONE',  ( 10.19999999999991047, 2.500000000000000000, -4.083716857408426826 ) ) ;
#35926=ORIENTED_EDGE ( 'NONE', *, *, #67383, .T. ) ;
#35927=EDGE_CURVE ( 'NONE', #102542, #64648, #18516, .T. ) ;
#35928=ORIENTED_EDGE ( 'NONE', *, *, #103554, .F. ) ;
#35929=EDGE_CURVE ( 'NONE', #65247, #1730, #30048, .T. ) ;
#35930=DIRECTION ( 'NONE',  ( -0.000000000000000000, -1.000000000000000000, -0.000000000000000000 ) ) ;
#35931=AXIS2_PLACEMENT_3D ( 'NONE', #68544, #118940, #17502 ) ;
#35932=ORIENTED_EDGE ( 'NONE', *, *, #1972, .F. ) ;
#35933=FACE_OUTER_BOUND ( 'NONE', #86767, .T. ) ;
#35934=VECTOR ( 'NONE', #15980, 1000.000000000000000 ) ;
#35935=FACE_OUTER_BOUND ( 'NONE', #20849, .T. ) ;
#35936=CIRCLE ( 'NONE', #52655, 0.1000000000000002554 ) ;
#35937=ORIENTED_EDGE ( 'NONE', *, *, #103662, .F. ) ;
#35938=AXIS2_PLACEMENT_3D ( 'NONE', #49964, #110148, #70229 ) ;
#35939=CARTESIAN_POINT ( 'NONE',  ( -11.44999999999999929, 2.500000000000000000, -1.818653347947322141 ) ) ;
#35940=CARTESIAN_POINT ( 'NONE',  ( -0.6500000000000389910, 2.500000000000000000, -6.048780366869526581 ) ) ;
#35941=CARTESIAN_POINT ( 'NONE',  ( -8.350000000000010303, 12.50000000000000000, 6.495190528383297135 ) ) ;
#35942=DIRECTION ( 'NONE',  ( 0.000000000000000000, 0.000000000000000000, 1.000000000000000000 ) ) ;
#35943=LINE ( 'NONE', #66680, #102975 ) ;
#35944=ADVANCED_FACE ( 'NONE', ( #27055 ), #46769, .T. ) ;
#35945=CARTESIAN_POINT ( 'NONE',  ( -6.850000000000017408, 12.50000000000000000, -6.148780366869526226 ) ) ;
#35946=CONICAL_SURFACE ( 'NONE', #100684, 0.1000000000000000472, 0.003490658503988666988 ) ;
#35947=ORIENTED_EDGE ( 'NONE', *, *, #53835, .F. ) ;
#35948=AXIS2_PLACEMENT_3D ( 'NONE', #101085, #11411, #90612 ) ;
#35949=ORIENTED_EDGE ( 'NONE', *, *, #108929, .F. ) ;
#35950=DIRECTION ( 'NONE',  ( -0.000000000000000000, -1.000000000000000000, -0.000000000000000000 ) ) ;
#35951=CARTESIAN_POINT ( 'NONE',  ( 16.70850060796086467, -0.4765610498145330665, 5.930927070179653704 ) ) ;
#35952=CIRCLE ( 'NONE', #81904, 0.1000000000000002554 ) ;
#35953=CONICAL_SURFACE ( 'NONE', #58943, 0.1000000000000000472, 0.003490658503988666988 ) ;
#35954=VECTOR ( 'NONE', #35146, 1000.000000000000000 ) ;
#35955=DIRECTION ( 'NONE',  ( 0.000000000000000000, 0.000000000000000000, -1.000000000000000000 ) ) ;
#35957=ORIENTED_EDGE ( 'NONE', *, *, #128872, .T. ) ;
#35958=ORIENTED_EDGE ( 'NONE', *, *, #35261, .F. ) ;
#35959=DIRECTION ( 'NONE',  ( 0.000000000000000000, -0.9999939076577903929, 0.003490651415223739937 ) ) ;
#35960=AXIS2_PLACEMENT_3D ( 'NONE', #4155, #76630, #44097 ) ;
#35961=DIRECTION ( 'NONE',  ( -0.000000000000000000, 1.000000000000000000, -0.000000000000000000 ) ) ;
#35962=CARTESIAN_POINT ( 'NONE',  ( 10.59999999999990905, 2.500000000000000000, 4.576537180435972019 ) ) ;
#35964=CARTESIAN_POINT ( 'NONE',  ( 9.599999999999917932, 2.500000000000000000, 0.09999999999999772959 ) ) ;
#35965=AXIS2_PLACEMENT_3D ( 'NONE', #123173, #61018, #91770 ) ;
#35966=CARTESIAN_POINT ( 'NONE',  ( 11.24999999999991118, 2.500000000000000000, -2.957883832488653830 ) ) ;
#35967=DIRECTION ( 'NONE',  ( 0.000000000000000000, 0.000000000000000000, 1.000000000000000000 ) ) ;
#35968=CARTESIAN_POINT ( 'NONE',  ( -5.400000000000019895, 12.50000000000000000, -2.276824562219559311E-15 ) ) ;
#35969=DIRECTION ( 'NONE',  ( -4.274815082592931898E-19, -0.9999939076577903929, -0.003490651415223739937 ) ) ;
#35970=LINE ( 'NONE', #75244, #14344 ) ;
#35971=ORIENTED_EDGE ( 'NONE', *, *, #112422, .F. ) ;
#35972=ADVANCED_FACE ( 'NONE', ( #128502 ), #58461, .T. ) ;
#35973=CARTESIAN_POINT ( 'NONE',  ( 9.199999999999919353, 2.500000000000000000, -0.1000000000000022815 ) ) ;
#35974=ORIENTED_EDGE ( 'NONE', *, *, #1075, .T. ) ;
#35975=ORIENTED_EDGE ( 'NONE', *, *, #116470, .T. ) ;
#35976=EDGE_CURVE ( 'NONE', #34456, #62695, #8671, .T. ) ;
#35977=DIRECTION ( 'NONE',  ( 0.000000000000000000, -0.000000000000000000, 1.000000000000000000 ) ) ;
#35978=DIRECTION ( 'NONE',  ( 0.000000000000000000, 0.000000000000000000, 1.000000000000000000 ) ) ;
#35979=DIRECTION ( 'NONE',  ( -0.000000000000000000, -1.000000000000000000, -0.000000000000000000 ) ) ;
#35980=EDGE_CURVE ( 'NONE', #2098, #36092, #9344, .T. ) ;
#35981=FACE_OUTER_BOUND ( 'NONE', #42247, .T. ) ;
#35982=FACE_OUTER_BOUND ( 'NONE', #107537, .T. ) ;
#35983=CARTESIAN_POINT ( 'NONE',  ( 9.799999999999918998, 2.500000000000000000, -0.4464101615137782142 ) ) ;
#35984=CIRCLE ( 'NONE', #109116, 0.1000000000000000472 ) ;
#35985=CARTESIAN_POINT ( 'NONE',  ( 2.499999999999948930, 2.500000000000000000, -0.5928203230275541635 ) ) ;
#35986=ORIENTED_EDGE ( 'NONE', *, *, #3988, .F. ) ;
#35987=CARTESIAN_POINT ( 'NONE',  ( 6.249999999999928946, 12.50000000000000000, 2.857883832488649301 ) ) ;
#35988=AXIS2_PLACEMENT_3D ( 'NONE', #100890, #68861, #99626 ) ;
#35989=EDGE_CURVE ( 'NONE', #41467, #115621, #13291, .T. ) ;
#35990=AXIS2_PLACEMENT_3D ( 'NONE', #56412, #38072, #66873 ) ;
#35991=EDGE_CURVE ( 'NONE', #49421, #89608, #63490, .T. ) ;
#35993=EDGE_CURVE ( 'NONE', #37339, #59274, #27676, .T. ) ;
#35994=CARTESIAN_POINT ( 'NONE',  ( -0.2000000000000339284, 12.50000000000000000, -0.3464101615137759604 ) ) ;
#35995=ORIENTED_EDGE ( 'NONE', *, *, #84446, .T. ) ;
#35996=AXIS2_PLACEMENT_3D ( 'NONE', #83377, #25088, #63735 ) ;
#35997=VERTEX_POINT ( 'NONE', #81935 ) ;
#35999=AXIS2_PLACEMENT_3D ( 'NONE', #19701, #59655, #49819 ) ;
#36000=ADVANCED_FACE ( 'NONE', ( #21750 ), #30936, .T. ) ;
#36001=ORIENTED_EDGE ( 'NONE', *, *, #28221, .T. ) ;
#36002=AXIS2_PLACEMENT_3D ( 'NONE', #23208, #43526, #36918 ) ;
#36003=CIRCLE ( 'NONE', #69437, 0.1000000000000002554 ) ;
#36004=EDGE_LOOP ( 'NONE', ( #39355, #67929, #67795, #5921 ) ) ;
#36005=FACE_OUTER_BOUND ( 'NONE', #89697, .T. ) ;
#36006=FACE_OUTER_BOUND ( 'NONE', #58103, .T. ) ;
#36007=EDGE_CURVE ( 'NONE', #61414, #88412, #50982, .T. ) ;
#36008=AXIS2_PLACEMENT_3D ( 'NONE', #12313, #32641, #43101 ) ;
#36009=DIRECTION ( 'NONE',  ( 0.000000000000000000, 0.000000000000000000, 1.000000000000000000 ) ) ;
#36010=DIRECTION ( 'NONE',  ( 0.000000000000000000, 1.000000000000000000, 0.000000000000000000 ) ) ;
#36011=CARTESIAN_POINT ( 'NONE',  ( 4.599999999999937472, 12.50000000000000000, 0.6277270498435120194 ) ) ;
#36012=ORIENTED_EDGE ( 'NONE', *, *, #67794, .T. ) ;
#36013=CARTESIAN_POINT ( 'NONE',  ( 3.749999999999978684, 12.50000000000000000, -2.230156782645139391 ) ) ;
#36014=CARTESIAN_POINT ( 'NONE',  ( -4.999999999999986677, 2.500000000000000000, 4.330127018922196314 ) ) ;
#36015=ORIENTED_EDGE ( 'NONE', *, *, #106305, .T. ) ;
#36016=ORIENTED_EDGE ( 'NONE', *, *, #63426, .F. ) ;
#36017=ORIENTED_EDGE ( 'NONE', *, *, #40467, .T. ) ;
#36018=DIRECTION ( 'NONE',  ( 0.000000000000000000, 1.000000000000000000, 0.000000000000000000 ) ) ;
#36019=CARTESIAN_POINT ( 'NONE',  ( -1.650000000000035216, 2.500000000000000000, -1.572243186433550211 ) ) ;
#36020=AXIS2_PLACEMENT_3D ( 'NONE', #69654, #40874, #1553 ) ;
#36021=LINE ( 'NONE', #125036, #92093 ) ;
#36022=VERTEX_POINT ( 'NONE', #81313 ) ;
#36023=CARTESIAN_POINT ( 'NONE',  ( 4.349999999999940137, 12.50000000000000000, -2.511473670974877948 ) ) ;
#36024=DIRECTION ( 'NONE',  ( 0.000000000000000000, 1.000000000000000000, 0.000000000000000000 ) ) ;
#36025=FACE_OUTER_BOUND ( 'NONE', #117748, .T. ) ;
#36026=DIRECTION ( 'NONE',  ( 0.000000000000000000, -0.000000000000000000, 1.000000000000000000 ) ) ;
#36027=CARTESIAN_POINT ( 'NONE',  ( -12.49999999999999289, 2.500000000000000000, 5.022947341949748790 ) ) ;
#36028=CIRCLE ( 'NONE', #123840, 0.06509327318403741736 ) ;
#36029=AXIS2_PLACEMENT_3D ( 'NONE', #77494, #38900, #97785 ) ;
#36030=CONICAL_SURFACE ( 'NONE', #23500, 0.1000000000000000472, 0.003490658503988666988 ) ;
#36031=ORIENTED_EDGE ( 'NONE', *, *, #118023, .T. ) ;
#36032=DIRECTION ( 'NONE',  ( 0.000000000000000000, 0.000000000000000000, 1.000000000000000000 ) ) ;
#36033=AXIS2_PLACEMENT_3D ( 'NONE', #101046, #51325, #91230 ) ;
#36034=EDGE_CURVE ( 'NONE', #51049, #50142, #32110, .T. ) ;
#36035=ORIENTED_EDGE ( 'NONE', *, *, #122180, .F. ) ;
#36036=ORIENTED_EDGE ( 'NONE', *, *, #123170, .T. ) ;
#36037=ORIENTED_EDGE ( 'NONE', *, *, #471, .T. ) ;
#36038=DIRECTION ( 'NONE',  ( 0.000000000000000000, 0.000000000000000000, -1.000000000000000000 ) ) ;
#36039=FACE_BOUND ( 'NONE', #42574, .T. ) ;
#36040=CARTESIAN_POINT ( 'NONE',  ( -9.400000000000007461, 2.500000000000000000, 3.983716857408420076 ) ) ;
#36041=CIRCLE ( 'NONE', #71539, 0.1000000000000002554 ) ;
#36042=LINE ( 'NONE', #55026, #79854 ) ;
#36043=AXIS2_PLACEMENT_3D ( 'NONE', #21737, #19800, #71461 ) ;
#36044=DIRECTION ( 'NONE',  ( 0.000000000000000000, 1.000000000000000000, 0.000000000000000000 ) ) ;
#36045=EDGE_CURVE ( 'NONE', #60753, #106745, #25833, .T. ) ;
#36046=AXIS2_PLACEMENT_3D ( 'NONE', #23563, #42584, #82502 ) ;
#36047=AXIS2_PLACEMENT_3D ( 'NONE', #121764, #119841, #100828 ) ;
#36048=AXIS2_PLACEMENT_3D ( 'NONE', #121901, #91800, #13220 ) ;
#36049=ORIENTED_EDGE ( 'NONE', *, *, #15701, .T. ) ;
#36050=PLANE ( 'NONE',  #33452 ) ;
#36051=CARTESIAN_POINT ( 'NONE',  ( -6.050000000000020250, 12.50000000000000000, -6.776507416713040577 ) ) ;
#36052=DIRECTION ( 'NONE',  ( 0.000000000000000000, -0.000000000000000000, 1.000000000000000000 ) ) ;
#36053=CIRCLE ( 'NONE', #94613, 0.06509327318403745899 ) ;
#36054=CARTESIAN_POINT ( 'NONE',  ( -0.6500000000000389910, 12.50000000000000000, -1.883746621131363597 ) ) ;
#36055=VERTEX_POINT ( 'NONE', #112707 ) ;
#36056=DIRECTION ( 'NONE',  ( 0.000000000000000000, 0.000000000000000000, -1.000000000000000000 ) ) ;
#36057=DIRECTION ( 'NONE',  ( 0.000000000000000000, 0.000000000000000000, 1.000000000000000000 ) ) ;
#36058=VECTOR ( 'NONE', #95482, 1000.000000000000000 ) ;
#36059=EDGE_LOOP ( 'NONE', ( #84541, #104760, #33414, #124802 ) ) ;
#36060=DIRECTION ( 'NONE',  ( 0.000000000000000000, 0.000000000000000000, 1.000000000000000000 ) ) ;
#36061=FACE_BOUND ( 'NONE', #12103, .T. ) ;
#36062=DIRECTION ( 'NONE',  ( 0.000000000000000000, -0.000000000000000000, 1.000000000000000000 ) ) ;
#36063=ORIENTED_EDGE ( 'NONE', *, *, #45022, .F. ) ;
#36064=PLANE ( 'NONE',  #121802 ) ;
#36065=DIRECTION ( 'NONE',  ( 0.000000000000000000, 1.000000000000000000, 0.000000000000000000 ) ) ;
#36066=EDGE_LOOP ( 'NONE', ( #115074, #66647 ) ) ;
#36067=ORIENTED_EDGE ( 'NONE', *, *, #101309, .T. ) ;
#36069=ORIENTED_EDGE ( 'NONE', *, *, #38758, .F. ) ;
#36071=DIRECTION ( 'NONE',  ( 0.000000000000000000, 0.000000000000000000, 1.000000000000000000 ) ) ;
#36072=ADVANCED_FACE ( 'NONE', ( #61014 ), #51220, .T. ) ;
#36073=VECTOR ( 'NONE', #32394, 1000.000000000000000 ) ;
#36074=CARTESIAN_POINT ( 'NONE',  ( -3.950000000000029932, 2.500000000000000000, -6.148780366869526226 ) ) ;
#36075=DIRECTION ( 'NONE',  ( 0.000000000000000000, 0.000000000000000000, -1.000000000000000000 ) ) ;
#36076=CIRCLE ( 'NONE', #119690, 0.1000000000000002554 ) ;
#36077=CARTESIAN_POINT ( 'NONE',  ( 14.39999999999989555, 2.500000000000000000, -0.3464101615137782364 ) ) ;
#36078=EDGE_CURVE ( 'NONE', #3072, #26527, #80221, .T. ) ;
#36079=VECTOR ( 'NONE', #42599, 1000.000000000000000 ) ;
#36080=VECTOR ( 'NONE', #10402, 1000.000000000000000 ) ;
#36081=ORIENTED_EDGE ( 'NONE', *, *, #74111, .F. ) ;
#36082=CARTESIAN_POINT ( 'NONE',  ( -9.350000000000006750, 12.50000000000000000, -2.511473670974877948 ) ) ;
#36083=DIRECTION ( 'NONE',  ( 0.000000000000000000, -0.9999939076577903929, 0.003490651415223739937 ) ) ;
#36084=LINE ( 'NONE', #66175, #99454 ) ;
#36085=VECTOR ( 'NONE', #99705, 1000.000000000000000 ) ;
#36086=CARTESIAN_POINT ( 'NONE',  ( -5.650000000000019895, 2.500000000000000000, 2.511473670974873507 ) ) ;
#36087=CONICAL_SURFACE ( 'NONE', #17176, 0.09999999999999982514, 0.003490658503988666988 ) ;
#36088=ORIENTED_EDGE ( 'NONE', *, *, #74212, .T. ) ;
#36089=VERTEX_POINT ( 'NONE', #111390 ) ;
#36090=ADVANCED_FACE ( 'NONE', ( #91127 ), #96918, .T. ) ;
#36091=FACE_OUTER_BOUND ( 'NONE', #35016, .T. ) ;
#36092=VERTEX_POINT ( 'NONE', #30297 ) ;
#36093=ADVANCED_FACE ( 'NONE', ( #61683 ), #80015, .T. ) ;
#36094=DIRECTION ( 'NONE',  ( 0.000000000000000000, 0.000000000000000000, -1.000000000000000000 ) ) ;
#36095=DIRECTION ( 'NONE',  ( 0.000000000000000000, 0.000000000000000000, 1.000000000000000000 ) ) ;
#36096=VECTOR ( 'NONE', #103123, 1000.000000000000000 ) ;
#36097=ORIENTED_EDGE ( 'NONE', *, *, #125059, .T. ) ;
#36098=CARTESIAN_POINT ( 'NONE',  ( 7.499999999999960032, 12.50000000000000000, -2.276824562219559311E-15 ) ) ;
#36099=CARTESIAN_POINT ( 'NONE',  ( 12.89999999999989910, 2.500000000000000000, 0.5928203230275495006 ) ) ;
#36100=CARTESIAN_POINT ( 'NONE',  ( 11.24999999999990763, 2.500000000000000000, 1.372243186433545370 ) ) ;
#36101=DIRECTION ( 'NONE',  ( 0.000000000000000000, 0.000000000000000000, -1.000000000000000000 ) ) ;
#36102=ORIENTED_EDGE ( 'NONE', *, *, #20618, .T. ) ;
#36103=EDGE_CURVE ( 'NONE', #90584, #115529, #32232, .T. ) ;
#36104=DIRECTION ( 'NONE',  ( 0.000000000000000000, 0.000000000000000000, -1.000000000000000000 ) ) ;
#36105=DIRECTION ( 'NONE',  ( 0.000000000000000000, 0.000000000000000000, 1.000000000000000000 ) ) ;
#36107=FACE_OUTER_BOUND ( 'NONE', #122428, .T. ) ;
#36108=EDGE_CURVE ( 'NONE', #4340, #87979, #11913, .T. ) ;
#36109=DIRECTION ( 'NONE',  ( -0.000000000000000000, -1.000000000000000000, -0.000000000000000000 ) ) ;
#36110=CONICAL_SURFACE ( 'NONE', #109247, 0.1000000000000002554, 0.003490658503988666988 ) ;
#36111=ORIENTED_EDGE ( 'NONE', *, *, #7111, .T. ) ;
#36112=ORIENTED_EDGE ( 'NONE', *, *, #14807, .F. ) ;
#36114=EDGE_LOOP ( 'NONE', ( #71242, #16864 ) ) ;
#36115=CARTESIAN_POINT ( 'NONE',  ( 16.55874544816223448, 0.4845305829267578801, 6.091953208799004926 ) ) ;
#36117=ORIENTED_EDGE ( 'NONE', *, *, #15399, .F. ) ;
#36118=VERTEX_POINT ( 'NONE', #148 ) ;
#36119=CARTESIAN_POINT ( 'NONE',  ( 3.099999999999945466, 2.500000000000000000, -3.983716857408426293 ) ) ;
#36120=AXIS2_PLACEMENT_3D ( 'NONE', #118754, #120693, #121330 ) ;
#36121=( GEOMETRIC_REPRESENTATION_CONTEXT ( 3 ) GLOBAL_UNCERTAINTY_ASSIGNED_CONTEXT ( ( #72987 ) ) GLOBAL_UNIT_ASSIGNED_CONTEXT ( ( #16004, #35040, #14064 ) ) REPRESENTATION_CONTEXT ( 'NONE', 'WORKASPACE' ) );
#36122=LINE ( 'NONE', #104836, #105312 ) ;
#36123=DIRECTION ( 'NONE',  ( -0.000000000000000000, -1.000000000000000000, -0.000000000000000000 ) ) ;
#36124=CARTESIAN_POINT ( 'NONE',  ( 13.94999999999989804, 2.500000000000000000, 1.918653347947321564 ) ) ;
#36125=CARTESIAN_POINT ( 'NONE',  ( 8.949999999999919353, 12.50000000000000000, 2.446380397790835826 ) ) ;
#36126=VERTEX_POINT ( 'NONE', #51857 ) ;
#36127=AXIS2_PLACEMENT_3D ( 'NONE', #93040, #13809, #54387 ) ;
#36128=AXIS2_PLACEMENT_3D ( 'NONE', #120976, #31326, #90869 ) ;
#36129=CARTESIAN_POINT ( 'NONE',  ( -2.499999999999996447, 2.500000000000000000, 4.230127018922196669 ) ) ;
#36130=EDGE_LOOP ( 'NONE', ( #21744, #77276 ) ) ;
#36131=VECTOR ( 'NONE', #67456, 1000.000000000000000 ) ;
#36132=EDGE_LOOP ( 'NONE', ( #15616, #114676, #117990, #44042 ) ) ;
#36133=ORIENTED_EDGE ( 'NONE', *, *, #98924, .T. ) ;
#36134=AXIS2_PLACEMENT_3D ( 'NONE', #20404, #89137, #90408 ) ;
#36135=EDGE_LOOP ( 'NONE', ( #123384, #90819, #3856, #23855 ) ) ;
#36136=CARTESIAN_POINT ( 'NONE',  ( -13.14999999999999147, 12.50000000000000000, 2.576566944158914740 ) ) ;
#36137=EDGE_LOOP ( 'NONE', ( #107114, #36930, #121102, #70757 ) ) ;
#36138=VERTEX_POINT ( 'NONE', #91768 ) ;
#36139=AXIS2_PLACEMENT_3D ( 'NONE', #71959, #113810, #122349 ) ;
#36140=CARTESIAN_POINT ( 'NONE',  ( -11.69999999999999929, 12.50000000000000000, -4.265033745738161741 ) ) ;
#36141=CARTESIAN_POINT ( 'NONE',  ( 4.199999999999939782, 2.500000000000000000, -2.276824562219559311E-15 ) ) ;
#36142=CARTESIAN_POINT ( 'NONE',  ( -1.250000000000036193, 2.500000000000000000, 5.902370205355745192 ) ) ;
#36143=AXIS2_PLACEMENT_3D ( 'NONE', #19304, #60559, #38329 ) ;
#36144=DIRECTION ( 'NONE',  ( 0.000000000000000000, 0.000000000000000000, 1.000000000000000000 ) ) ;
#36145=CIRCLE ( 'NONE', #117669, 0.06509327318403745899 ) ;
#36146=AXIS2_PLACEMENT_3D ( 'NONE', #80546, #103401, #110634 ) ;
#36147=EDGE_CURVE ( 'NONE', #13514, #63649, #113656, .T. ) ;
#36148=DIRECTION ( 'NONE',  ( 0.000000000000000000, 0.000000000000000000, 1.000000000000000000 ) ) ;
#36149=ORIENTED_EDGE ( 'NONE', *, *, #97974, .F. ) ;
#36150=ADVANCED_FACE ( 'NONE', ( #110123 ), #73949, .T. ) ;
#36151=CIRCLE ( 'NONE', #56951, 0.06509327318403745899 ) ;
#36152=EDGE_CURVE ( 'NONE', #54054, #79693, #90670, .T. ) ;
#36153=DIRECTION ( 'NONE',  ( 0.000000000000000000, -0.000000000000000000, 1.000000000000000000 ) ) ;
#36154=EDGE_CURVE ( 'NONE', #111830, #31107, #72140, .T. ) ;
#36155=VERTEX_POINT ( 'NONE', #90463 ) ;
#36156=DIRECTION ( 'NONE',  ( 0.000000000000000000, 1.000000000000000000, 0.000000000000000000 ) ) ;
#36157=EDGE_LOOP ( 'NONE', ( #126404, #108385, #117041, #55018 ) ) ;
#36158=AXIS2_PLACEMENT_3D ( 'NONE', #10939, #79709, #12246 ) ;
#36159=CARTESIAN_POINT ( 'NONE',  ( -8.550000000000013145, 2.500000000000000000, 2.511473670974873507 ) ) ;
#36160=EDGE_CURVE ( 'NONE', #104949, #17389, #17492, .T. ) ;
#36161=VERTEX_POINT ( 'NONE', #121871 ) ;
#36162=ORIENTED_EDGE ( 'NONE', *, *, #40193, .T. ) ;
#36163=FACE_OUTER_BOUND ( 'NONE', #50120, .T. ) ;
#36164=DIRECTION ( 'NONE',  ( 0.000000000000000000, -0.000000000000000000, 1.000000000000000000 ) ) ;
#36165=EDGE_CURVE ( 'NONE', #86890, #71724, #61448, .T. ) ;
#36166=ADVANCED_FACE ( 'NONE', ( #115239 ), #88510, .T. ) ;
#36168=CARTESIAN_POINT ( 'NONE',  ( -1.250000000000035749, 12.50000000000000000, -7.253104124594891289 ) ) ;
#36169=CARTESIAN_POINT ( 'NONE',  ( -6.250000000000017764, 2.500000000000000000, 7.288010851410849256 ) ) ;
#36170=VERTEX_POINT ( 'NONE', #26260 ) ;
#36171=CARTESIAN_POINT ( 'NONE',  ( -8.750000000000008882, 12.50000000000000000, 1.472243186433545459 ) ) ;
#36172=DIRECTION ( 'NONE',  ( 0.000000000000000000, 1.000000000000000000, 0.000000000000000000 ) ) ;
#36173=CONICAL_SURFACE ( 'NONE', #29900, 0.09999999999999999167, 0.003490658503988666988 ) ;
#36174=AXIS2_PLACEMENT_3D ( 'NONE', #73993, #105386, #44529 ) ;
#36175=DIRECTION ( 'NONE',  ( 0.000000000000000000, 0.000000000000000000, 1.000000000000000000 ) ) ;
#36176=CARTESIAN_POINT ( 'NONE',  ( -11.64999999999999680, 2.500000000000000000, 7.188010851410848723 ) ) ;
#36177=PLANE ( 'NONE',  #62585 ) ;
#36178=EDGE_LOOP ( 'NONE', ( #82732, #124968 ) ) ;
#36179=AXIS2_PLACEMENT_3D ( 'NONE', #79024, #99300, #111693 ) ;
#36180=VECTOR ( 'NONE', #100763, 1000.000000000000000 ) ;
#36181=ORIENTED_EDGE ( 'NONE', *, *, #40226, .T. ) ;
#36182=VECTOR ( 'NONE', #49648, 1000.000000000000000 ) ;
#36183=AXIS2_PLACEMENT_3D ( 'NONE', #127281, #27767, #17281 ) ;
#36184=DIRECTION ( 'NONE',  ( 0.000000000000000000, 1.000000000000000000, 0.000000000000000000 ) ) ;
#36185=ORIENTED_EDGE ( 'NONE', *, *, #52568, .F. ) ;
#36186=CARTESIAN_POINT ( 'NONE',  ( -6.650000000000019007, 12.50000000000000000, -5.802370205355749988 ) ) ;
#36187=FACE_OUTER_BOUND ( 'NONE', #15313, .T. ) ;
#36188=CONICAL_SURFACE ( 'NONE', #50844, 0.1000000000000000472, 0.003490658503988666988 ) ;
#36189=CIRCLE ( 'NONE', #34127, 0.06509327318403745899 ) ;
#36190=AXIS2_PLACEMENT_3D ( 'NONE', #127291, #104415, #87336 ) ;
#36191=VECTOR ( 'NONE', #119015, 1000.000000000000000 ) ;
#36192=AXIS2_PLACEMENT_3D ( 'NONE', #71877, #50951, #82343 ) ;
#36193=VERTEX_POINT ( 'NONE', #24960 ) ;
#36195=CARTESIAN_POINT ( 'NONE',  ( 0.5999999999999555689, 2.500000000000000000, 4.776537180435972196 ) ) ;
#36196=DIRECTION ( 'NONE',  ( -4.274815082592931898E-19, -0.9999939076577903929, -0.003490651415223739937 ) ) ;
#36197=DIRECTION ( 'NONE',  ( 0.000000000000000000, 0.000000000000000000, -1.000000000000000000 ) ) ;
#36198=ORIENTED_EDGE ( 'NONE', *, *, #24759, .T. ) ;
#36199=AXIS2_PLACEMENT_3D ( 'NONE', #87813, #26990, #26345 ) ;
#36200=PLANE ( 'NONE',  #375 ) ;
#36201=LINE ( 'NONE', #13958, #55972 ) ;
#36202=EDGE_LOOP ( 'NONE', ( #83443, #3376 ) ) ;
#36205=DIRECTION ( 'NONE',  ( -0.000000000000000000, -1.000000000000000000, -0.000000000000000000 ) ) ;
#36206=AXIS2_PLACEMENT_3D ( 'NONE', #38133, #66298, #75470 ) ;
#36207=EDGE_CURVE ( 'NONE', #55939, #4440, #84408, .T. ) ;
#36208=ORIENTED_EDGE ( 'NONE', *, *, #37325, .T. ) ;
#36209=LINE ( 'NONE', #58428, #109606 ) ;
#36210=ORIENTED_EDGE ( 'NONE', *, *, #5937, .T. ) ;
#36211=LINE ( 'NONE', #89163, #35404 ) ;
#36212=CARTESIAN_POINT ( 'NONE',  ( -9.350000000000006750, 2.500000000000000000, 2.611473670974873151 ) ) ;
#36213=CARTESIAN_POINT ( 'NONE',  ( -12.49999999999999289, 12.50000000000000000, 5.022947341949748790 ) ) ;
#36214=CONICAL_SURFACE ( 'NONE', #2735, 0.09999999999999982514, 0.003490658503988666988 ) ;
#36215=ORIENTED_EDGE ( 'NONE', *, *, #35919, .T. ) ;
#36217=AXIS2_PLACEMENT_3D ( 'NONE', #77286, #127675, #79868 ) ;
#36218=CARTESIAN_POINT ( 'NONE',  ( 6.249999999999930722, 2.500000000000000000, 7.088010851410848190 ) ) ;
#36219=DIRECTION ( 'NONE',  ( 0.000000000000000000, 0.000000000000000000, -1.000000000000000000 ) ) ;
#36220=EDGE_LOOP ( 'NONE', ( #39395, #66330, #82392, #70243 ) ) ;
#36221=ORIENTED_EDGE ( 'NONE', *, *, #11522, .T. ) ;
#36222=CONICAL_SURFACE ( 'NONE', #126085, 0.1000000000000002554, 0.003490658503988666988 ) ;
#36223=FACE_OUTER_BOUND ( 'NONE', #65100, .T. ) ;
#36224=AXIS2_PLACEMENT_3D ( 'NONE', #121729, #25966, #46238 ) ;
#36225=AXIS2_PLACEMENT_3D ( 'NONE', #60342, #117942, #69486 ) ;
#36226=EDGE_LOOP ( 'NONE', ( #5655, #108563 ) ) ;
#36227=LINE ( 'NONE', #37518, #2481 ) ;
#36228=DIRECTION ( 'NONE',  ( 0.000000000000000000, 1.000000000000000000, 0.000000000000000000 ) ) ;
#36229=ORIENTED_EDGE ( 'NONE', *, *, #110080, .F. ) ;
#36230=CARTESIAN_POINT ( 'NONE',  ( -4.350000000000023626, 2.500000000000000000, 6.841600689897072485 ) ) ;
#36231=CARTESIAN_POINT ( 'NONE',  ( 13.34999999999990017, 2.500000000000000000, 2.265063509461097357 ) ) ;
#36232=CIRCLE ( 'NONE', #19489, 0.1000000000000002554 ) ;
#36233=VERTEX_POINT ( 'NONE', #63606 ) ;
#36234=DIRECTION ( 'NONE',  ( -0.000000000000000000, -1.000000000000000000, -0.000000000000000000 ) ) ;
#36235=FACE_OUTER_BOUND ( 'NONE', #49503, .T. ) ;
#36236=CIRCLE ( 'NONE', #11174, 0.09999999999999982514 ) ;
#36237=CIRCLE ( 'NONE', #73880, 0.06509327318403745899 ) ;
#36238=AXIS2_PLACEMENT_3D ( 'NONE', #37872, #117697, #8400 ) ;
#36239=DIRECTION ( 'NONE',  ( 0.000000000000000000, 0.000000000000000000, -1.000000000000000000 ) ) ;
#36240=LINE ( 'NONE', #94486, #82176 ) ;
#36241=CARTESIAN_POINT ( 'NONE',  ( 6.449999999999933564, 12.50000000000000000, -6.841600689897078702 ) ) ;
#36242=AXIS2_PLACEMENT_3D ( 'NONE', #6265, #44269, #105124 ) ;
#36243=CARTESIAN_POINT ( 'NONE',  ( -12.09999999999999609, 2.500000000000000000, 4.330127018922196314 ) ) ;
#36244=EDGE_CURVE ( 'NONE', #52125, #76693, #64239, .T. ) ;
#36245=EDGE_CURVE ( 'NONE', #14798, #86952, #101144, .T. ) ;
#36246=ORIENTED_EDGE ( 'NONE', *, *, #117163, .T. ) ;
#36247=ORIENTED_EDGE ( 'NONE', *, *, #107368, .T. ) ;
#36248=ORIENTED_EDGE ( 'NONE', *, *, #94990, .T. ) ;
#36249=ORIENTED_EDGE ( 'NONE', *, *, #60271, .F. ) ;
#36250=DIRECTION ( 'NONE',  ( 0.000000000000000000, -0.9999939076577903929, 0.003490651415223739937 ) ) ;
#36251=CARTESIAN_POINT ( 'NONE',  ( -5.000000000000023093, 12.50000000000000000, 0.6928203230275494784 ) ) ;
#36252=DIRECTION ( 'NONE',  ( -0.000000000000000000, 1.000000000000000000, -0.000000000000000000 ) ) ;
#36254=EDGE_CURVE ( 'NONE', #86066, #107157, #105244, .T. ) ;
#36255=FACE_BOUND ( 'NONE', #30367, .T. ) ;
#36256=EDGE_CURVE ( 'NONE', #89857, #82534, #125718, .T. ) ;
#36257=DIRECTION ( 'NONE',  ( 0.000000000000000000, -0.9999939076577903929, 0.003490651415223739937 ) ) ;
#36258=DIRECTION ( 'NONE',  ( -4.274815082592931898E-19, -0.9999939076577903929, -0.003490651415223739937 ) ) ;
#36259=DIRECTION ( 'NONE',  ( 0.000000000000000000, 1.000000000000000000, 0.000000000000000000 ) ) ;
#36261=CARTESIAN_POINT ( 'NONE',  ( 8.549999999999918998, 12.50000000000000000, 6.841600689897072485 ) ) ;
#36262=EDGE_CURVE ( 'NONE', #29188, #9068, #19571, .T. ) ;
#36263=CARTESIAN_POINT ( 'NONE',  ( 8.349999999999919709, 12.50000000000000000, 5.802370205355744659 ) ) ;
#36264=EDGE_CURVE ( 'NONE', #40264, #31157, #36317, .T. ) ;
#36265=DIRECTION ( 'NONE',  ( -0.000000000000000000, -1.000000000000000000, -0.000000000000000000 ) ) ;
#36266=CARTESIAN_POINT ( 'NONE',  ( 12.89999999999990266, 2.500000000000000000, 3.637306695894644726 ) ) ;
#36267=CIRCLE ( 'NONE', #40474, 0.1000000000000002554 ) ;
#36268=EDGE_CURVE ( 'NONE', #48509, #108123, #35439, .T. ) ;
#36269=CARTESIAN_POINT ( 'NONE',  ( -13.34999999999999076, 2.500000000000000000, 2.857883832488652853 ) ) ;
#36270=ADVANCED_FACE ( 'NONE', ( #83252 ), #97023, .T. ) ;
#36271=ADVANCED_FACE ( 'NONE', ( #75991 ), #55068, .T. ) ;
#36272=DIRECTION ( 'NONE',  ( 0.000000000000000000, 1.000000000000000000, 0.000000000000000000 ) ) ;
#36273=CIRCLE ( 'NONE', #63448, 0.06509327318403745899 ) ;
#36274=CONICAL_SURFACE ( 'NONE', #40485, 0.1000000000000002554, 0.003490658503988666988 ) ;
#36275=ORIENTED_EDGE ( 'NONE', *, *, #93721, .T. ) ;
#36276=ORIENTED_EDGE ( 'NONE', *, *, #100392, .F. ) ;
#36277=ORIENTED_EDGE ( 'NONE', *, *, #71746, .T. ) ;
#36278=AXIS2_PLACEMENT_3D ( 'NONE', #9013, #107223, #28677 ) ;
#36279=ORIENTED_EDGE ( 'NONE', *, *, #122846, .F. ) ;
#36280=DIRECTION ( 'NONE',  ( 0.000000000000000000, 0.000000000000000000, 1.000000000000000000 ) ) ;
#36281=ORIENTED_EDGE ( 'NONE', *, *, #123019, .F. ) ;
#36282=VECTOR ( 'NONE', #93155, 1000.000000000000000 ) ;
#36283=CARTESIAN_POINT ( 'NONE',  ( 12.93920187831608892, 1.500000000000000444, -10.00000000000000000 ) ) ;
#36284=ORIENTED_EDGE ( 'NONE', *, *, #52247, .F. ) ;
#36285=EDGE_CURVE ( 'NONE', #61216, #48774, #38563, .T. ) ;
#36286=ORIENTED_EDGE ( 'NONE', *, *, #20763, .F. ) ;
#36287=DIRECTION ( 'NONE',  ( 0.000000000000000000, 0.000000000000000000, 1.000000000000000000 ) ) ;
#36288=AXIS2_PLACEMENT_3D ( 'NONE', #16347, #26197, #56287 ) ;
#36289=CIRCLE ( 'NONE', #126148, 0.06509327318403745899 ) ;
#36290=VECTOR ( 'NONE', #50036, 1000.000000000000000 ) ;
#36292=CARTESIAN_POINT ( 'NONE',  ( 2.500000000000002220, -2.500000000000000444, 10.00000000000000178 ) ) ;
#36293=DIRECTION ( 'NONE',  ( -4.274815082592931898E-19, -0.9999939076577903929, -0.003490651415223739937 ) ) ;
#36294=CARTESIAN_POINT ( 'NONE',  ( 12.09999999999990550, 12.50000000000000000, -5.022947341949754119 ) ) ;
#36295=CIRCLE ( 'NONE', #86430, 0.06509327318403745899 ) ;
#36296=DIRECTION ( 'NONE',  ( 0.000000000000000000, 1.000000000000000000, 0.000000000000000000 ) ) ;
#36297=CIRCLE ( 'NONE', #61319, 0.06509327318403743123 ) ;
#36298=VERTEX_POINT ( 'NONE', #5308 ) ;
#36299=VERTEX_POINT ( 'NONE', #113334 ) ;
#36301=ORIENTED_EDGE ( 'NONE', *, *, #126260, .F. ) ;
#36302=DIRECTION ( 'NONE',  ( -0.000000000000000000, -1.000000000000000000, -0.000000000000000000 ) ) ;
#36303=ORIENTED_EDGE ( 'NONE', *, *, #2274, .F. ) ;
#36304=VERTEX_POINT ( 'NONE', #15774 ) ;
#36305=VECTOR ( 'NONE', #45228, 1000.000000000000000 ) ;
#36306=DIRECTION ( 'NONE',  ( 0.000000000000000000, 0.000000000000000000, 1.000000000000000000 ) ) ;
#36307=CARTESIAN_POINT ( 'NONE',  ( -5.200000000000022382, 2.500000000000000000, 4.576537180435972019 ) ) ;
#36308=DIRECTION ( 'NONE',  ( 0.000000000000000000, 0.000000000000000000, 1.000000000000000000 ) ) ;
#36309=CARTESIAN_POINT ( 'NONE',  ( -1.250000000000001554, 12.50000000000000000, 6.495190528383297135 ) ) ;
#36310=LINE ( 'NONE', #13416, #12619 ) ;
#36311=DIRECTION ( 'NONE',  ( -4.274815082592931898E-19, -0.9999939076577903929, -0.003490651415223739937 ) ) ;
#36312=EDGE_CURVE ( 'NONE', #40294, #68357, #105345, .T. ) ;
#36313=CONICAL_SURFACE ( 'NONE', #23676, 0.1000000000000000472, 0.003490658503988666988 ) ;
#36314=EDGE_LOOP ( 'NONE', ( #1930, #113902, #22307, #16619 ) ) ;
#36315=EDGE_CURVE ( 'NONE', #85897, #75229, #99093, .T. ) ;
#36316=DIRECTION ( 'NONE',  ( 0.000000000000000000, -0.9999939076577903929, 0.003490651415223739937 ) ) ;
#36317=CIRCLE ( 'NONE', #126276, 0.1000000000000000472 ) ;
#36318=VECTOR ( 'NONE', #42001, 1000.000000000000000 ) ;
#36319=VERTEX_POINT ( 'NONE', #95638 ) ;
#36320=CARTESIAN_POINT ( 'NONE',  ( 0.5999999999999547917, 2.500000000000000000, 3.883716857408420431 ) ) ;
#36321=EDGE_CURVE ( 'NONE', #77871, #82944, #48920, .T. ) ;
#36322=ORIENTED_EDGE ( 'NONE', *, *, #74269, .F. ) ;
#36323=DIRECTION ( 'NONE',  ( 0.000000000000000000, 0.000000000000000000, -1.000000000000000000 ) ) ;
#36324=CARTESIAN_POINT ( 'NONE',  ( -14.54999999999998472, 12.50000000000000000, -2.165063509461099489 ) ) ;
#36326=DIRECTION ( 'NONE',  ( 0.000000000000000000, 0.000000000000000000, -1.000000000000000000 ) ) ;
#36327=EDGE_CURVE ( 'NONE', #37524, #27204, #74041, .T. ) ;
#36328=CARTESIAN_POINT ( 'NONE',  ( 3.749999999999976907, 2.500000000000000000, 2.065063509461097624 ) ) ;
#36329=CIRCLE ( 'NONE', #44724, 0.06509327318403745899 ) ;
#36330=ORIENTED_EDGE ( 'NONE', *, *, #32287, .F. ) ;
#36331=ADVANCED_FACE ( 'NONE', ( #93074 ), #46860, .T. ) ;
#36332=CIRCLE ( 'NONE', #115713, 0.1000000000000000472 ) ;
#36333=EDGE_CURVE ( 'NONE', #17919, #7073, #32310, .T. ) ;
#36334=AXIS2_PLACEMENT_3D ( 'NONE', #62270, #73354, #12502 ) ;
#36335=EDGE_CURVE ( 'NONE', #127093, #110872, #10320, .T. ) ;
#36336=CARTESIAN_POINT ( 'NONE',  ( 9.549999999999915445, 12.50000000000000000, -2.165063509461101710 ) ) ;
#36337=VERTEX_POINT ( 'NONE', #46521 ) ;
#36338=ORIENTED_EDGE ( 'NONE', *, *, #59850, .T. ) ;
#36339=CARTESIAN_POINT ( 'NONE',  ( 8.099999999999923261, 2.500000000000000000, 4.576537180435972019 ) ) ;
#36340=FACE_OUTER_BOUND ( 'NONE', #53450, .T. ) ;
#36342=AXIS2_PLACEMENT_3D ( 'NONE', #116252, #37708, #35148 ) ;
#36344=EDGE_CURVE ( 'NONE', #63527, #104908, #71992, .T. ) ;
#36345=DIRECTION ( 'NONE',  ( 0.000000000000000000, 1.000000000000000000, 0.000000000000000000 ) ) ;
#36346=AXIS2_PLACEMENT_3D ( 'NONE', #98990, #29600, #70180 ) ;
#36347=CONICAL_SURFACE ( 'NONE', #73881, 0.1000000000000002554, 0.003490658503988666988 ) ;
#36348=CARTESIAN_POINT ( 'NONE',  ( 9.599999999999914380, 12.50000000000000000, -5.022947341949754119 ) ) ;
#36349=CIRCLE ( 'NONE', #84349, 0.09999999999999982514 ) ;
#36350=ORIENTED_EDGE ( 'NONE', *, *, #60815, .T. ) ;
#36351=CIRCLE ( 'NONE', #92772, 0.06509327318403745899 ) ;
#36352=CARTESIAN_POINT ( 'NONE',  ( -1.650000000000034328, 2.500000000000000000, -6.495190528383302464 ) ) ;
#36353=ORIENTED_EDGE ( 'NONE', *, *, #23441, .F. ) ;
#36354=DIRECTION ( 'NONE',  ( 0.000000000000000000, 0.000000000000000000, 1.000000000000000000 ) ) ;
#36355=EDGE_CURVE ( 'NONE', #78070, #90721, #129480, .T. ) ;
#36356=PLANE ( 'NONE',  #73655 ) ;
#36357=DIRECTION ( 'NONE',  ( -4.274815082592931898E-19, -0.9999939076577903929, -0.003490651415223739937 ) ) ;
#36358=ORIENTED_EDGE ( 'NONE', *, *, #73394, .F. ) ;
#36359=CARTESIAN_POINT ( 'NONE',  ( 12.04999999999990834, 12.50000000000000000, -2.099970236277064473 ) ) ;
#36360=DIRECTION ( 'NONE',  ( -4.274815082592931898E-19, -0.9999939076577903929, -0.003490651415223739937 ) ) ;
#36361=AXIS2_PLACEMENT_3D ( 'NONE', #12293, #24065, #121601 ) ;
#36362=EDGE_LOOP ( 'NONE', ( #127268, #21059, #16395, #30662 ) ) ;
#36363=FACE_OUTER_BOUND ( 'NONE', #9043, .T. ) ;
#36364=AXIS2_PLACEMENT_3D ( 'NONE', #123287, #32993, #92530 ) ;
#36365=AXIS2_PLACEMENT_3D ( 'NONE', #89441, #91372, #30546 ) ;
#36366=EDGE_CURVE ( 'NONE', #107907, #44142, #88708, .T. ) ;
#36367=ORIENTED_EDGE ( 'NONE', *, *, #17438, .T. ) ;
#36368=ORIENTED_EDGE ( 'NONE', *, *, #119197, .T. ) ;
#36369=CARTESIAN_POINT ( 'NONE',  ( -2.950000000000033484, 12.50000000000000000, -6.495190528383302464 ) ) ;
#36370=VECTOR ( 'NONE', #94543, 1000.000000000000000 ) ;
#36371=ORIENTED_EDGE ( 'NONE', *, *, #31744, .F. ) ;
#36372=CARTESIAN_POINT ( 'NONE',  ( 12.89999999999990266, 2.500000000000000000, -3.537306695894649966 ) ) ;
#36373=DIRECTION ( 'NONE',  ( -0.000000000000000000, 1.000000000000000000, -0.000000000000000000 ) ) ;
#36374=DIRECTION ( 'NONE',  ( 0.000000000000000000, 0.000000000000000000, -1.000000000000000000 ) ) ;
#36375=AXIS2_PLACEMENT_3D ( 'NONE', #30734, #70630, #11047 ) ;
#36376=EDGE_LOOP ( 'NONE', ( #80683, #65530 ) ) ;
#36377=VECTOR ( 'NONE', #26163, 1000.000000000000000 ) ;
#36378=FACE_BOUND ( 'NONE', #80539, .T. ) ;
#36379=CARTESIAN_POINT ( 'NONE',  ( -11.64999999999999680, 2.500000000000000000, -6.495190528383298911 ) ) ;
#36381=AXIS2_PLACEMENT_3D ( 'NONE', #123693, #34721, #114529 ) ;
#36382=DIRECTION ( 'NONE',  ( -0.000000000000000000, -1.000000000000000000, -0.000000000000000000 ) ) ;
#36383=EDGE_CURVE ( 'NONE', #55213, #14119, #56344, .T. ) ;
#36384=DIRECTION ( 'NONE',  ( 0.000000000000000000, 0.000000000000000000, 1.000000000000000000 ) ) ;
#36386=VERTEX_POINT ( 'NONE', #90811 ) ;
#36387=ORIENTED_EDGE ( 'NONE', *, *, #34396, .T. ) ;
#36388=DIRECTION ( 'NONE',  ( -0.000000000000000000, 1.000000000000000000, -0.000000000000000000 ) ) ;
#36389=FACE_OUTER_BOUND ( 'NONE', #115900, .T. ) ;
#36390=CARTESIAN_POINT ( 'NONE',  ( -4.150000000000024336, 2.500000000000000000, 1.472243186433545459 ) ) ;
#36391=FACE_BOUND ( 'NONE', #73501, .T. ) ;
#36392=ORIENTED_EDGE ( 'NONE', *, *, #3023, .T. ) ;
#36394=DIRECTION ( 'NONE',  ( 0.000000000000000000, -0.9999939076577903929, 0.003490651415223739937 ) ) ;
#36395=CARTESIAN_POINT ( 'NONE',  ( -5.450000000000019718, 2.500000000000000000, 6.495190528383297135 ) ) ;
#36396=AXIS2_PLACEMENT_3D ( 'NONE', #49753, #48439, #18966 ) ;
#36397=CARTESIAN_POINT ( 'NONE',  ( 1.699999999999951994, 12.50000000000000000, -4.395220292106239768 ) ) ;
#36398=DIRECTION ( 'NONE',  ( -0.000000000000000000, -1.000000000000000000, -0.000000000000000000 ) ) ;
#36399=DIRECTION ( 'NONE',  ( 0.000000000000000000, -0.000000000000000000, 1.000000000000000000 ) ) ;
#36400=DIRECTION ( 'NONE',  ( 0.000000000000000000, 1.000000000000000000, 0.000000000000000000 ) ) ;
#36401=CARTESIAN_POINT ( 'NONE',  ( 12.69999999999990337, 2.500000000000000000, -4.676537180435978769 ) ) ;
#36402=AXIS2_PLACEMENT_3D ( 'NONE', #106102, #16399, #96259 ) ;
#36403=AXIS2_PLACEMENT_3D ( 'NONE', #62299, #72116, #102217 ) ;
#36404=CARTESIAN_POINT ( 'NONE',  ( 8.349999999999919709, 2.500000000000000000, -2.165063509461101710 ) ) ;
#36405=EDGE_CURVE ( 'NONE', #122680, #119243, #63582, .T. ) ;
#36406=VERTEX_POINT ( 'NONE', #41095 ) ;
#36407=ORIENTED_EDGE ( 'NONE', *, *, #82452, .F. ) ;
#36408=ORIENTED_EDGE ( 'NONE', *, *, #28169, .F. ) ;
#36409=EDGE_LOOP ( 'NONE', ( #34937, #53870, #103938, #13561 ) ) ;
#36410=ORIENTED_EDGE ( 'NONE', *, *, #112470, .T. ) ;
#36411=CARTESIAN_POINT ( 'NONE',  ( -9.800000000000006040, 2.500000000000000000, 0.2464101615137735679 ) ) ;
#36412=DIRECTION ( 'NONE',  ( -4.274815082592931898E-19, -0.9999939076577903929, -0.003490651415223739937 ) ) ;
#36413=ORIENTED_EDGE ( 'NONE', *, *, #93211, .F. ) ;
#36414=FACE_BOUND ( 'NONE', #37277, .T. ) ;
#36415=AXIS2_PLACEMENT_3D ( 'NONE', #18175, #40423, #30604 ) ;
#36416=DIRECTION ( 'NONE',  ( -0.000000000000000000, -1.000000000000000000, -0.000000000000000000 ) ) ;
#36417=AXIS2_PLACEMENT_3D ( 'NONE', #68951, #67653, #87924 ) ;
#36418=CARTESIAN_POINT ( 'NONE',  ( 14.14999999999989200, 12.50000000000000000, -2.165063509461101710 ) ) ;
#36419=ADVANCED_FACE ( 'NONE', ( #100615 ), #53119, .T. ) ;
#36420=CARTESIAN_POINT ( 'NONE',  ( 1.249999999999952038, 12.50000000000000000, 2.857883832488649301 ) ) ;
#36421=ADVANCED_FACE ( 'NONE', ( #120281 ), #103296, .T. ) ;
#36422=CARTESIAN_POINT ( 'NONE',  ( 14.14999999999989733, 2.500000000000000000, 2.857883832488649301 ) ) ;
#36423=EDGE_CURVE ( 'NONE', #5118, #107, #7123, .T. ) ;
#36424=DIRECTION ( 'NONE',  ( 0.000000000000000000, 1.000000000000000000, 0.000000000000000000 ) ) ;
#36425=EDGE_CURVE ( 'NONE', #30237, #18179, #86553, .T. ) ;
#36426=ORIENTED_EDGE ( 'NONE', *, *, #22588, .T. ) ;
#36427=CARTESIAN_POINT ( 'NONE',  ( 16.88398462908939024, -2.500000000000000000, 4.430583899596162389 ) ) ;
#36428=VERTEX_POINT ( 'NONE', #79074 ) ;
#36429=VECTOR ( 'NONE', #45234, 1000.000000000000000 ) ;
#36430=AXIS2_PLACEMENT_3D ( 'NONE', #12405, #92924, #90976 ) ;
#36431=AXIS2_PLACEMENT_3D ( 'NONE', #117980, #9970, #109457 ) ;
#36432=ORIENTED_EDGE ( 'NONE', *, *, #36007, .T. ) ;
#36433=ORIENTED_EDGE ( 'NONE', *, *, #68518, .T. ) ;
#36434=CARTESIAN_POINT ( 'NONE',  ( -10.60000000000000142, 2.500000000000000000, 0.4464101615137736623 ) ) ;
#36435=DIRECTION ( 'NONE',  ( -0.000000000000000000, 1.000000000000000000, -0.000000000000000000 ) ) ;
#36436=FACE_OUTER_BOUND ( 'NONE', #81082, .T. ) ;
#36437=AXIS2_PLACEMENT_3D ( 'NONE', #106266, #114159, #84691 ) ;
#36438=ORIENTED_EDGE ( 'NONE', *, *, #6779, .F. ) ;
#36439=EDGE_CURVE ( 'NONE', #119031, #22231, #51071, .T. ) ;
#36440=CARTESIAN_POINT ( 'NONE',  ( 16.31260002278204979, 1.500000000000484945, -6.357732714000876584 ) ) ;
#36441=AXIS2_PLACEMENT_3D ( 'NONE', #3059, #90782, #10902 ) ;
#36442=EDGE_CURVE ( 'NONE', #76941, #93392, #20789, .T. ) ;
#36443=CARTESIAN_POINT ( 'NONE',  ( 14.59999999999989484, 12.50000000000000000, -0.7579135962115916003 ) ) ;
#36444=EDGE_CURVE ( 'NONE', #84243, #73744, #30141, .T. ) ;
#36445=DIRECTION ( 'NONE',  ( -0.000000000000000000, -1.000000000000000000, -0.000000000000000000 ) ) ;
#36447=CARTESIAN_POINT ( 'NONE',  ( 11.04999999999991189, 12.50000000000000000, 6.148780366869520897 ) ) ;
#36448=DIRECTION ( 'NONE',  ( 0.000000000000000000, -0.000000000000000000, 1.000000000000000000 ) ) ;
#36449=ORIENTED_EDGE ( 'NONE', *, *, #80789, .T. ) ;
#36450=DIRECTION ( 'NONE',  ( 0.000000000000000000, 0.000000000000000000, 1.000000000000000000 ) ) ;
#36451=ORIENTED_EDGE ( 'NONE', *, *, #58566, .F. ) ;
#36452=CIRCLE ( 'NONE', #1208, 0.1000000000000002554 ) ;
#36453=ORIENTED_EDGE ( 'NONE', *, *, #12295, .T. ) ;
#36454=DIRECTION ( 'NONE',  ( 0.000000000000000000, 0.000000000000000000, 1.000000000000000000 ) ) ;
#36455=AXIS2_PLACEMENT_3D ( 'NONE', #83646, #101354, #52251 ) ;
#36457=CARTESIAN_POINT ( 'NONE',  ( 7.949999999999922018, 2.500000000000000000, -2.065063509461102065 ) ) ;
#36458=CARTESIAN_POINT ( 'NONE',  ( 8.749999999999918288, 2.500000000000000000, -1.572243186433550211 ) ) ;
#36459=ORIENTED_EDGE ( 'NONE', *, *, #22663, .T. ) ;
#36460=ORIENTED_EDGE ( 'NONE', *, *, #47799, .F. ) ;
#36461=CARTESIAN_POINT ( 'NONE',  ( 11.64999999999990798, 12.50000000000000000, 7.188010851410848723 ) ) ;
#36462=CIRCLE ( 'NONE', #107448, 0.06509327318403745899 ) ;
#36463=CONICAL_SURFACE ( 'NONE', #92795, 0.1000000000000002554, 0.003490658503988666988 ) ;
#36464=VECTOR ( 'NONE', #63061, 1000.000000000000000 ) ;
#36465=DIRECTION ( 'NONE',  ( 0.000000000000000000, 0.000000000000000000, -1.000000000000000000 ) ) ;
#36466=CARTESIAN_POINT ( 'NONE',  ( 1.249999999999988454, 12.50000000000000000, 2.165063509461097713 ) ) ;
#36467=ORIENTED_EDGE ( 'NONE', *, *, #63327, .T. ) ;
#36468=ORIENTED_EDGE ( 'NONE', *, *, #57850, .F. ) ;
#36469=DIRECTION ( 'NONE',  ( 0.000000000000000000, -0.9999939076577903929, 0.003490651415223739937 ) ) ;
#36470=ORIENTED_EDGE ( 'NONE', *, *, #16294, .F. ) ;
#36471=CARTESIAN_POINT ( 'NONE',  ( 8.549999999999920774, 2.500000000000000000, -2.511473670974877948 ) ) ;
#36472=AXIS2_PLACEMENT_3D ( 'NONE', #67887, #108456, #59395 ) ;
#36473=VECTOR ( 'NONE', #56877, 1000.000000000000000 ) ;
#36474=AXIS2_PLACEMENT_3D ( 'NONE', #67424, #79229, #57649 ) ;
#36475=PLANE ( 'NONE',  #88854 ) ;
#36477=CARTESIAN_POINT ( 'NONE',  ( -0.6000000000000323963, 12.50000000000000000, -0.3464101615137759604 ) ) ;
#36478=DIRECTION ( 'NONE',  ( 0.000000000000000000, 1.000000000000000000, 0.000000000000000000 ) ) ;
#36479=DIRECTION ( 'NONE',  ( -0.000000000000000000, -1.000000000000000000, -0.000000000000000000 ) ) ;
#36480=EDGE_CURVE ( 'NONE', #84566, #75902, #67773, .T. ) ;
#36481=CARTESIAN_POINT ( 'NONE',  ( -5.600000000000020073, 12.50000000000000000, -0.3464101615137782364 ) ) ;
#36482=ORIENTED_EDGE ( 'NONE', *, *, #54469, .F. ) ;
#36483=EDGE_CURVE ( 'NONE', #110257, #57396, #90757, .T. ) ;
#36484=DIRECTION ( 'NONE',  ( -4.274815082592931898E-19, -0.9999939076577903929, -0.003490651415223739937 ) ) ;
#36485=LINE ( 'NONE', #107118, #39499 ) ;
#36486=ADVANCED_FACE ( 'NONE', ( #26900 ), #66800, .T. ) ;
#36487=ORIENTED_EDGE ( 'NONE', *, *, #99287, .F. ) ;
#36488=ORIENTED_EDGE ( 'NONE', *, *, #37937, .F. ) ;
#36490=FACE_OUTER_BOUND ( 'NONE', #72358, .T. ) ;
#36491=DIRECTION ( 'NONE',  ( 0.000000000000000000, -0.9999939076577903929, 0.003490651415223739937 ) ) ;
#36492=FACE_OUTER_BOUND ( 'NONE', #69605, .T. ) ;
#36493=VECTOR ( 'NONE', #123250, 1000.000000000000000 ) ;
#36494=CARTESIAN_POINT ( 'NONE',  ( 7.499999999999961808, 2.500000000000000000, -4.230127018922201998 ) ) ;
#36495=EDGE_CURVE ( 'NONE', #18083, #61323, #7234, .T. ) ;
#36496=DIRECTION ( 'NONE',  ( 0.000000000000000000, 0.000000000000000000, 1.000000000000000000 ) ) ;
#36497=FACE_OUTER_BOUND ( 'NONE', #104976, .T. ) ;
#36498=CARTESIAN_POINT ( 'NONE',  ( -8.750000000000012434, 12.50000000000000000, -5.802370205355744659 ) ) ;
#36499=DIRECTION ( 'NONE',  ( 0.000000000000000000, 0.000000000000000000, -1.000000000000000000 ) ) ;
#36500=CARTESIAN_POINT ( 'NONE',  ( 14.34999999999989662, 2.500000000000000000, 2.511473670974873507 ) ) ;
#36501=CONICAL_SURFACE ( 'NONE', #109644, 0.1000000000000002554, 0.003490658503988666988 ) ;
#36502=EDGE_LOOP ( 'NONE', ( #105730, #69787 ) ) ;
#36503=CONICAL_SURFACE ( 'NONE', #32311, 0.09999999999999982514, 0.003490658503988666988 ) ;
#36504=ORIENTED_EDGE ( 'NONE', *, *, #86080, .T. ) ;
#36505=DIRECTION ( 'NONE',  ( -0.000000000000000000, -1.000000000000000000, -0.000000000000000000 ) ) ;
#36506=EDGE_LOOP ( 'NONE', ( #39226, #52185 ) ) ;
#36507=DIRECTION ( 'NONE',  ( 0.000000000000000000, 1.000000000000000000, 0.000000000000000000 ) ) ;
#36508=DIRECTION ( 'NONE',  ( 0.000000000000000000, 1.000000000000000000, 0.000000000000000000 ) ) ;
#36509=DIRECTION ( 'NONE',  ( 0.000000000000000000, 1.000000000000000000, 0.000000000000000000 ) ) ;
#36510=EDGE_LOOP ( 'NONE', ( #19281, #123579 ) ) ;
#36511=FACE_OUTER_BOUND ( 'NONE', #27255, .T. ) ;
#36512=AXIS2_PLACEMENT_3D ( 'NONE', #87732, #127667, #8521 ) ;
#36514=LINE ( 'NONE', #54830, #56417 ) ;
#36515=ORIENTED_EDGE ( 'NONE', *, *, #74204, .T. ) ;
#36516=DIRECTION ( 'NONE',  ( 0.000000000000000000, 0.000000000000000000, 1.000000000000000000 ) ) ;
#36518=AXIS2_PLACEMENT_3D ( 'NONE', #1912, #21568, #70030 ) ;
#36520=EDGE_CURVE ( 'NONE', #58017, #92342, #32206, .T. ) ;
#36521=ORIENTED_EDGE ( 'NONE', *, *, #16460, .T. ) ;
#36522=VERTEX_POINT ( 'NONE', #111069 ) ;
#36523=EDGE_LOOP ( 'NONE', ( #106441, #107156 ) ) ;
#36525=CONICAL_SURFACE ( 'NONE', #103320, 0.1000000000000002554, 0.003490658503988666988 ) ;
#36526=DIRECTION ( 'NONE',  ( 0.000000000000000000, 1.000000000000000000, 0.000000000000000000 ) ) ;
#36527=FACE_OUTER_BOUND ( 'NONE', #75274, .T. ) ;
#36528=CIRCLE ( 'NONE', #15563, 0.1000000000000002554 ) ;
#36529=DIRECTION ( 'NONE',  ( -0.000000000000000000, -1.000000000000000000, -0.000000000000000000 ) ) ;
#36530=ORIENTED_EDGE ( 'NONE', *, *, #44447, .F. ) ;
#36531=DIRECTION ( 'NONE',  ( -4.274815082592931898E-19, -0.9999939076577903929, -0.003490651415223739937 ) ) ;
#36532=ADVANCED_FACE ( 'NONE', ( #103862 ), #19662, .T. ) ;
#36533=EDGE_LOOP ( 'NONE', ( #73395, #34139 ) ) ;
#36534=CARTESIAN_POINT ( 'NONE',  ( 43.06166283093421043, -3.066941195868620351, -4.904920240848436030 ) ) ;
#36535=DIRECTION ( 'NONE',  ( 0.000000000000000000, 0.000000000000000000, 1.000000000000000000 ) ) ;
#36536=FACE_OUTER_BOUND ( 'NONE', #11455, .T. ) ;
#36537=CARTESIAN_POINT ( 'NONE',  ( 19.51231976789167888, -0.5900868802299801263, 4.348342248683190192 ) ) ;
#36538=EDGE_CURVE ( 'NONE', #41232, #25471, #78263, .T. ) ;
#36539=VERTEX_POINT ( 'NONE', #3713 ) ;
#36540=ORIENTED_EDGE ( 'NONE', *, *, #122149, .T. ) ;
#36541=CONICAL_SURFACE ( 'NONE', #111737, 0.1000000000000002554, 0.003490658503988666988 ) ;
#36542=ORIENTED_EDGE ( 'NONE', *, *, #70111, .F. ) ;
#36543=CARTESIAN_POINT ( 'NONE',  ( -5.450000000000023270, 2.500000000000000000, -2.165063509461101710 ) ) ;
#36544=DIRECTION ( 'NONE',  ( -0.000000000000000000, -1.000000000000000000, -0.000000000000000000 ) ) ;
#36545=AXIS2_PLACEMENT_3D ( 'NONE', #106331, #124032, #16638 ) ;
#36546=VECTOR ( 'NONE', #68444, 1000.000000000000000 ) ;
#36547=EDGE_CURVE ( 'NONE', #92822, #89168, #113679, .T. ) ;
#36548=DIRECTION ( 'NONE',  ( 0.000000000000000000, -0.000000000000000000, 1.000000000000000000 ) ) ;
#36549=FACE_BOUND ( 'NONE', #38075, .T. ) ;
#36550=DIRECTION ( 'NONE',  ( 0.000000000000000000, 1.000000000000000000, 0.000000000000000000 ) ) ;
#36551=FACE_OUTER_BOUND ( 'NONE', #115487, .T. ) ;
#36552=CARTESIAN_POINT ( 'NONE',  ( 1.049999999999954081, 12.50000000000000000, -6.083687093685488989 ) ) ;
#36553=CARTESIAN_POINT ( 'NONE',  ( -7.700000000000014388, 12.50000000000000000, -0.3464101615137782364 ) ) ;
#36554=AXIS2_PLACEMENT_3D ( 'NONE', #74570, #26120, #114487 ) ;
#36555=AXIS2_PLACEMENT_3D ( 'NONE', #45489, #15990, #55929 ) ;
#36557=VECTOR ( 'NONE', #79635, 1000.000000000000000 ) ;
#36558=DIRECTION ( 'NONE',  ( 0.000000000000000000, -0.9999939076577903929, 0.003490651415223739937 ) ) ;
#36559=FACE_OUTER_BOUND ( 'NONE', #25541, .T. ) ;
#36560=CIRCLE ( 'NONE', #72144, 0.06509327318403745899 ) ;
#36561=VECTOR ( 'NONE', #40615, 1000.000000000000000 ) ;
#36562=DIRECTION ( 'NONE',  ( 0.000000000000000000, 0.000000000000000000, 1.000000000000000000 ) ) ;
#36563=ADVANCED_FACE ( 'NONE', ( #124132 ), #2949, .T. ) ;
#36564=ORIENTED_EDGE ( 'NONE', *, *, #33932, .F. ) ;
#36565=EDGE_LOOP ( 'NONE', ( #128480, #45498 ) ) ;
#36566=ORIENTED_EDGE ( 'NONE', *, *, #2706, .T. ) ;
#36567=ORIENTED_EDGE ( 'NONE', *, *, #124733, .T. ) ;
#36568=AXIS2_PLACEMENT_3D ( 'NONE', #4402, #82372, #5070 ) ;
#36569=DIRECTION ( 'NONE',  ( -0.000000000000000000, -1.000000000000000000, -0.000000000000000000 ) ) ;
#36570=FACE_BOUND ( 'NONE', #78323, .T. ) ;
#36571=CARTESIAN_POINT ( 'NONE',  ( -8.150000000000012790, 12.50000000000000000, -1.753560074763288679 ) ) ;
#36572=DIRECTION ( 'NONE',  ( 0.000000000000000000, 0.000000000000000000, -1.000000000000000000 ) ) ;
#36573=EDGE_CURVE ( 'NONE', #122182, #67250, #128444, .T. ) ;
#36574=ORIENTED_EDGE ( 'NONE', *, *, #95360, .T. ) ;
#36575=ADVANCED_FACE ( 'NONE', ( #4332 ), #41735, .T. ) ;
#36576=CARTESIAN_POINT ( 'NONE',  ( 0.6499999999999561684, 2.500000000000000000, -2.511473670974877948 ) ) ;
#36577=ADVANCED_FACE ( 'NONE', ( #1771 ), #92755, .T. ) ;
#36578=DIRECTION ( 'NONE',  ( 0.000000000000000000, 1.000000000000000000, 0.000000000000000000 ) ) ;
#36579=ADVANCED_FACE ( 'NONE', ( #102553 ), #54110, .T. ) ;
#36580=EDGE_CURVE ( 'NONE', #8551, #16094, #42772, .T. ) ;
#36581=AXIS2_PLACEMENT_3D ( 'NONE', #36251, #46066, #126559 ) ;
#36582=EDGE_LOOP ( 'NONE', ( #73348, #32390, #84064, #107464 ) ) ;
#36583=CARTESIAN_POINT ( 'NONE',  ( -4.800000000000024691, 12.50000000000000000, 4.611443907251934426 ) ) ;
#36584=CARTESIAN_POINT ( 'NONE',  ( -1.850000000000033396, 2.500000000000000000, -6.841600689897077814 ) ) ;
#36585=ADVANCED_FACE ( 'NONE', ( #21422 ), #40708, .T. ) ;
#36587=DIRECTION ( 'NONE',  ( 0.000000000000000000, 1.000000000000000000, 0.000000000000000000 ) ) ;
#36588=EDGE_CURVE ( 'NONE', #92462, #84837, #80406, .T. ) ;
#36589=DIRECTION ( 'NONE',  ( -4.274815082592931898E-19, -0.9999939076577903929, -0.003490651415223739937 ) ) ;
#36590=AXIS2_PLACEMENT_3D ( 'NONE', #60701, #118961, #48950 ) ;
#36591=EDGE_CURVE ( 'NONE', #4806, #84139, #126364, .T. ) ;
#36592=ORIENTED_EDGE ( 'NONE', *, *, #52247, .T. ) ;
#36593=CARTESIAN_POINT ( 'NONE',  ( -2.100000000000033396, 2.500000000000000000, -3.537306695894649966 ) ) ;
#36594=EDGE_CURVE ( 'NONE', #89245, #91598, #57414, .T. ) ;
#36595=CARTESIAN_POINT ( 'NONE',  ( 5.849999999999933920, 12.50000000000000000, 5.737276932171707422 ) ) ;
#36597=DIRECTION ( 'NONE',  ( 0.000000000000000000, 0.000000000000000000, -1.000000000000000000 ) ) ;
#36598=ORIENTED_EDGE ( 'NONE', *, *, #9699, .F. ) ;
#36599=ORIENTED_EDGE ( 'NONE', *, *, #6268, .F. ) ;
#36600=ADVANCED_FACE ( 'NONE', ( #91452 ), #38653, .T. ) ;
#36601=CARTESIAN_POINT ( 'NONE',  ( 6.899999999999926636, 2.500000000000000000, -0.3464101615137782364 ) ) ;
#36602=EDGE_CURVE ( 'NONE', #88265, #93018, #83584, .T. ) ;
#36603=EDGE_LOOP ( 'NONE', ( #123187, #101783, #21429, #71995 ) ) ;
#36604=DIRECTION ( 'NONE',  ( 0.000000000000000000, 0.000000000000000000, -1.000000000000000000 ) ) ;
#36605=CARTESIAN_POINT ( 'NONE',  ( -2.050000000000033129, 2.500000000000000000, 2.065063509461097624 ) ) ;
#36606=VECTOR ( 'NONE', #30901, 1000.000000000000000 ) ;
#36607=ORIENTED_EDGE ( 'NONE', *, *, #60109, .F. ) ;
#36608=DIRECTION ( 'NONE',  ( -0.000000000000000000, 1.000000000000000000, -0.000000000000000000 ) ) ;
#36609=FACE_OUTER_BOUND ( 'NONE', #64717, .T. ) ;
#36610=DIRECTION ( 'NONE',  ( 0.000000000000000000, 1.000000000000000000, 0.000000000000000000 ) ) ;
#36611=CARTESIAN_POINT ( 'NONE',  ( -6.650000000000014566, 2.500000000000000000, 2.065063509461097624 ) ) ;
#36612=DIRECTION ( 'NONE',  ( 0.000000000000000000, 1.000000000000000000, 0.000000000000000000 ) ) ;
#36613=DIRECTION ( 'NONE',  ( 0.000000000000000000, 0.000000000000000000, 1.000000000000000000 ) ) ;
#36614=ORIENTED_EDGE ( 'NONE', *, *, #110015, .T. ) ;
#36615=ORIENTED_EDGE ( 'NONE', *, *, #39849, .F. ) ;
#36616=FACE_OUTER_BOUND ( 'NONE', #39133, .T. ) ;
#36617=AXIS2_PLACEMENT_3D ( 'NONE', #90628, #59263, #99175 ) ;
#36618=DIRECTION ( 'NONE',  ( -4.274815082592931898E-19, -0.9999939076577903929, -0.003490651415223739937 ) ) ;
#36619=DIRECTION ( 'NONE',  ( 0.000000000000000000, 0.000000000000000000, 1.000000000000000000 ) ) ;
#36620=EDGE_LOOP ( 'NONE', ( #17534, #429, #21031, #86754 ) ) ;
#36622=ORIENTED_EDGE ( 'NONE', *, *, #114309, .F. ) ;
#36623=CARTESIAN_POINT ( 'NONE',  ( -5.600000000000023626, 2.500000000000000000, -3.983716857408426293 ) ) ;
#36624=CARTESIAN_POINT ( 'NONE',  ( 4.399999999999940847, 2.500000000000000000, -4.676537180435977881 ) ) ;
#36625=DIRECTION ( 'NONE',  ( 0.000000000000000000, 0.000000000000000000, 1.000000000000000000 ) ) ;
#36627=CARTESIAN_POINT ( 'NONE',  ( -9.350000000000006750, 2.500000000000000000, -2.511473670974877948 ) ) ;
#36628=LINE ( 'NONE', #37264, #56470 ) ;
#36629=DIRECTION ( 'NONE',  ( 0.000000000000000000, 1.000000000000000000, 0.000000000000000000 ) ) ;
#36630=CARTESIAN_POINT ( 'NONE',  ( 1.249999999999953815, 12.50000000000000000, 1.407149913249508000 ) ) ;
#36631=DIRECTION ( 'NONE',  ( -0.000000000000000000, -1.000000000000000000, -0.000000000000000000 ) ) ;
#36632=CIRCLE ( 'NONE', #74270, 0.1000000000000002554 ) ;
#36633=DIRECTION ( 'NONE',  ( 0.000000000000000000, 0.000000000000000000, -1.000000000000000000 ) ) ;
#36634=ORIENTED_EDGE ( 'NONE', *, *, #67973, .F. ) ;
#36635=EDGE_CURVE ( 'NONE', #53209, #41131, #23960, .T. ) ;
#36636=AXIS2_PLACEMENT_3D ( 'NONE', #40276, #90653, #29808 ) ;
#36637=CIRCLE ( 'NONE', #82696, 0.1000000000000002554 ) ;
#36638=ADVANCED_FACE ( 'NONE', ( #35761 ), #74141, .T. ) ;
#36639=CARTESIAN_POINT ( 'NONE',  ( 4.149999999999939959, 2.500000000000000000, 1.472243186433545459 ) ) ;
#36640=CIRCLE ( 'NONE', #28305, 0.09999999999999982514 ) ;
#36641=VERTEX_POINT ( 'NONE', #45589 ) ;
#36642=ORIENTED_EDGE ( 'NONE', *, *, #29798, .T. ) ;
#36643=CARTESIAN_POINT ( 'NONE',  ( -0.6000000000000388356, 2.500000000000000000, 4.676537180435972552 ) ) ;
#36644=DIRECTION ( 'NONE',  ( -4.274815082592931898E-19, -0.9999939076577903929, -0.003490651415223739937 ) ) ;
#36645=DIRECTION ( 'NONE',  ( 0.000000000000000000, 1.000000000000000000, 0.000000000000000000 ) ) ;
#36646=CIRCLE ( 'NONE', #120159, 0.09999999999999982514 ) ;
#36648=AXIS2_PLACEMENT_3D ( 'NONE', #3110, #32588, #92112 ) ;
#36650=FACE_OUTER_BOUND ( 'NONE', #84029, .T. ) ;
#36651=CARTESIAN_POINT ( 'NONE',  ( -4.600000000000025402, 2.500000000000000000, -0.1000000000000023925 ) ) ;
#36652=ORIENTED_EDGE ( 'NONE', *, *, #118124, .T. ) ;
#36653=DIRECTION ( 'NONE',  ( -0.000000000000000000, 1.000000000000000000, -0.000000000000000000 ) ) ;
#36654=AXIS2_PLACEMENT_3D ( 'NONE', #67876, #96677, #116967 ) ;
#36655=DIRECTION ( 'NONE',  ( 0.000000000000000000, 1.000000000000000000, 0.000000000000000000 ) ) ;
#36656=CIRCLE ( 'NONE', #126522, 0.1000000000000002554 ) ;
#36657=EDGE_LOOP ( 'NONE', ( #7278, #113874, #110452, #115694 ) ) ;
#36658=AXIS2_PLACEMENT_3D ( 'NONE', #40938, #56816, #40274 ) ;
#36659=EDGE_LOOP ( 'NONE', ( #34942, #98969 ) ) ;
#36660=ORIENTED_EDGE ( 'NONE', *, *, #69446, .T. ) ;
#36661=VERTEX_POINT ( 'NONE', #6910 ) ;
#36664=PLANE ( 'NONE',  #28965 ) ;
#36665=ORIENTED_EDGE ( 'NONE', *, *, #2797, .T. ) ;
#36666=CARTESIAN_POINT ( 'NONE',  ( -9.400000000000009237, 2.500000000000000000, -4.776537180435973973 ) ) ;
#36667=DIRECTION ( 'NONE',  ( -4.274815082592931898E-19, -0.9999939076577903929, -0.003490651415223739937 ) ) ;
#36668=CARTESIAN_POINT ( 'NONE',  ( -10.40000000000000213, 12.50000000000000000, -2.276824562219559311E-15 ) ) ;
#36669=ORIENTED_EDGE ( 'NONE', *, *, #11639, .F. ) ;
#36670=FACE_OUTER_BOUND ( 'NONE', #113950, .T. ) ;
#36671=AXIS2_PLACEMENT_3D ( 'NONE', #127050, #104799, #105470 ) ;
#36672=CARTESIAN_POINT ( 'NONE',  ( 4.999999999999935163, 2.500000000000000000, 0.7928203230275495672 ) ) ;
#36673=EDGE_CURVE ( 'NONE', #92388, #31556, #14792, .T. ) ;
#36674=ORIENTED_EDGE ( 'NONE', *, *, #83785, .T. ) ;
#36675=ORIENTED_EDGE ( 'NONE', *, *, #31422, .F. ) ;
#36676=EDGE_LOOP ( 'NONE', ( #28514, #72336 ) ) ;
#36677=DIRECTION ( 'NONE',  ( 0.000000000000000000, 0.000000000000000000, -1.000000000000000000 ) ) ;
#36678=CONICAL_SURFACE ( 'NONE', #63854, 0.1000000000000002554, 0.003490658503988666988 ) ;
#36679=CONICAL_SURFACE ( 'NONE', #109822, 0.1000000000000000472, 0.003490658503988666988 ) ;
#36680=DIRECTION ( 'NONE',  ( 0.000000000000000000, 0.000000000000000000, 1.000000000000000000 ) ) ;
#36682=VERTEX_POINT ( 'NONE', #46877 ) ;
#36683=CARTESIAN_POINT ( 'NONE',  ( 12.04999999999990479, 12.50000000000000000, 2.230156782645134950 ) ) ;
#36684=CARTESIAN_POINT ( 'NONE',  ( 0.3999999999999555023, 2.500000000000000000, 4.330127018922196314 ) ) ;
#36685=CARTESIAN_POINT ( 'NONE',  ( -5.800000000000018474, 2.500000000000000000, 4.330127018922196314 ) ) ;
#36686=DIRECTION ( 'NONE',  ( 0.000000000000000000, 0.000000000000000000, 1.000000000000000000 ) ) ;
#36687=EDGE_CURVE ( 'NONE', #82798, #75397, #67863, .T. ) ;
#36688=CIRCLE ( 'NONE', #84697, 0.06509327318403745899 ) ;
#36689=ORIENTED_EDGE ( 'NONE', *, *, #109582, .F. ) ;
#36690=DIRECTION ( 'NONE',  ( 0.000000000000000000, -0.000000000000000000, 1.000000000000000000 ) ) ;
#36691=AXIS2_PLACEMENT_3D ( 'NONE', #67264, #107228, #17548 ) ;
#36692=ORIENTED_EDGE ( 'NONE', *, *, #101131, .T. ) ;
#36693=EDGE_LOOP ( 'NONE', ( #58638, #7277, #76172, #51177 ) ) ;
#36694=VERTEX_POINT ( 'NONE', #25946 ) ;
#36695=ADVANCED_FACE ( 'NONE', ( #75665 ), #26023, .T. ) ;
#36696=CARTESIAN_POINT ( 'NONE',  ( -3.300000000000027800, 2.500000000000000000, -4.230127018922201998 ) ) ;
#36697=FACE_BOUND ( 'NONE', #122090, .T. ) ;
#36699=CARTESIAN_POINT ( 'NONE',  ( 1.849999999999949685, 12.50000000000000000, 1.753560074763284016 ) ) ;
#36700=CARTESIAN_POINT ( 'NONE',  ( -3.350000000000028955, 2.500000000000000000, -2.265063509461101798 ) ) ;
#36701=CONICAL_SURFACE ( 'NONE', #112004, 0.09999999999999982514, 0.003490658503988666988 ) ;
#36702=CONICAL_SURFACE ( 'NONE', #124529, 0.1000000000000000472, 0.003490658503988666988 ) ;
#36703=EDGE_LOOP ( 'NONE', ( #90753, #41753, #79156, #65612 ) ) ;
#36704=PLANE ( 'NONE',  #48105 ) ;
#36705=CARTESIAN_POINT ( 'NONE',  ( 6.249999999999932498, 12.50000000000000000, -2.857883832488653741 ) ) ;
#36706=CARTESIAN_POINT ( 'NONE',  ( 7.899999999999923084, 2.500000000000000000, 0.7928203230275495672 ) ) ;
#36707=CARTESIAN_POINT ( 'NONE',  ( 4.149999999999939959, 2.500000000000000000, -2.165063509461101710 ) ) ;
#36708=EDGE_LOOP ( 'NONE', ( #94960, #68030 ) ) ;
#36709=CARTESIAN_POINT ( 'NONE',  ( -6.250000000000017764, 2.500000000000000000, 2.757883832488649656 ) ) ;
#36710=DIRECTION ( 'NONE',  ( 0.000000000000000000, 0.000000000000000000, 1.000000000000000000 ) ) ;
#36711=CONICAL_SURFACE ( 'NONE', #126590, 0.1000000000000002554, 0.003490658503988666988 ) ;
#36712=EDGE_LOOP ( 'NONE', ( #2304, #44984 ) ) ;
#36713=LINE ( 'NONE', #87074, #43922 ) ;
#36714=CARTESIAN_POINT ( 'NONE',  ( -10.85000000000000142, 12.50000000000000000, -1.472243186433546125 ) ) ;
#36715=FACE_BOUND ( 'NONE', #40382, .T. ) ;
#36716=LINE ( 'NONE', #58288, #45180 ) ;
#36717=EDGE_CURVE ( 'NONE', #96763, #52365, #21916, .T. ) ;
#36718=CONICAL_SURFACE ( 'NONE', #11662, 0.1000000000000002554, 0.003490658503988666988 ) ;
#36719=ORIENTED_EDGE ( 'NONE', *, *, #65041, .T. ) ;
#36720=CARTESIAN_POINT ( 'NONE',  ( -0.4000000000000392131, 2.500000000000000000, -4.430127018922202176 ) ) ;
#36721=DIRECTION ( 'NONE',  ( -0.000000000000000000, -1.000000000000000000, -0.000000000000000000 ) ) ;
#36722=CIRCLE ( 'NONE', #51402, 0.06509327318403745899 ) ;
#36723=ORIENTED_EDGE ( 'NONE', *, *, #115878, .T. ) ;
#36724=VERTEX_POINT ( 'NONE', #75042 ) ;
#36725=EDGE_CURVE ( 'NONE', #31609, #22180, #90856, .T. ) ;
#36727=ADVANCED_FACE ( 'NONE', ( #125429 ), #3035, .T. ) ;
#36728=ORIENTED_EDGE ( 'NONE', *, *, #72215, .T. ) ;
#36730=CARTESIAN_POINT ( 'NONE',  ( 8.149999999999923972, 2.500000000000000000, 2.611473670974873151 ) ) ;
#36731=DIRECTION ( 'NONE',  ( 0.000000000000000000, 0.000000000000000000, 1.000000000000000000 ) ) ;
#36732=EDGE_CURVE ( 'NONE', #46460, #42124, #78352, .T. ) ;
#36733=ADVANCED_FACE ( 'NONE', ( #57333 ), #116875, .T. ) ;
#36734=DIRECTION ( 'NONE',  ( -0.000000000000000000, -1.000000000000000000, -0.000000000000000000 ) ) ;
#36735=ADVANCED_FACE ( 'NONE', ( #66495 ), #34491, .T. ) ;
#36736=CIRCLE ( 'NONE', #70178, 0.06509327318403745899 ) ;
#36737=VECTOR ( 'NONE', #30955, 1000.000000000000000 ) ;
#36739=CIRCLE ( 'NONE', #63917, 0.1000000000000000056 ) ;
#36740=DIRECTION ( 'NONE',  ( 0.000000000000000000, 0.000000000000000000, 1.000000000000000000 ) ) ;
#36741=ADVANCED_FACE ( 'NONE', ( #96589 ), #86782, .T. ) ;
#36742=CARTESIAN_POINT ( 'NONE',  ( 12.04999999999990479, 12.50000000000000000, -6.560283801567339701 ) ) ;
#36743=CARTESIAN_POINT ( 'NONE',  ( -4.800000000000026468, 2.500000000000000000, -4.776537180435978414 ) ) ;
#36744=AXIS2_PLACEMENT_3D ( 'NONE', #75921, #24252, #34740 ) ;
#36745=LINE ( 'NONE', #68109, #107323 ) ;
#36746=VERTEX_POINT ( 'NONE', #107059 ) ;
#36747=DIRECTION ( 'NONE',  ( 0.000000000000000000, 1.000000000000000000, 0.000000000000000000 ) ) ;
#36748=ORIENTED_EDGE ( 'NONE', *, *, #89628, .F. ) ;
#36749=DIRECTION ( 'NONE',  ( 0.000000000000000000, 1.000000000000000000, 0.000000000000000000 ) ) ;
#36750=CARTESIAN_POINT ( 'NONE',  ( 1.649999999999951505, 2.500000000000000000, 2.757883832488649656 ) ) ;
#36751=EDGE_CURVE ( 'NONE', #48843, #38503, #92925, .T. ) ;
#36752=ORIENTED_EDGE ( 'NONE', *, *, #126846, .F. ) ;
#36753=PLANE ( 'NONE',  #38909 ) ;
#36754=CARTESIAN_POINT ( 'NONE',  ( 87.49999999999998579, -4.871203238224193655, -5.733266569811711122 ) ) ;
#36755=DIRECTION ( 'NONE',  ( -4.274815082592931898E-19, -0.9999939076577903929, -0.003490651415223739937 ) ) ;
#36756=CARTESIAN_POINT ( 'NONE',  ( -11.84999999999999609, 2.500000000000000000, 6.941600689897073018 ) ) ;
#36757=ORIENTED_EDGE ( 'NONE', *, *, #126600, .T. ) ;
#36758=DIRECTION ( 'NONE',  ( 0.000000000000000000, 0.000000000000000000, -1.000000000000000000 ) ) ;
#36759=DIRECTION ( 'NONE',  ( -4.274815082592931898E-19, -0.9999939076577903929, -0.003490651415223739937 ) ) ;
#36761=DIRECTION ( 'NONE',  ( -0.000000000000000000, -1.000000000000000000, -0.000000000000000000 ) ) ;
#36762=VECTOR ( 'NONE', #29489, 1000.000000000000000 ) ;
#36763=PLANE ( 'NONE',  #116292 ) ;
#36764=ORIENTED_EDGE ( 'NONE', *, *, #88281, .F. ) ;
#36765=ORIENTED_EDGE ( 'NONE', *, *, #73106, .T. ) ;
#36766=CARTESIAN_POINT ( 'NONE',  ( -13.34999999999999076, 12.50000000000000000, 1.472243186433549456 ) ) ;
#36767=ORIENTED_EDGE ( 'NONE', *, *, #75759, .T. ) ;
#36768=CARTESIAN_POINT ( 'NONE',  ( 2.499999999999947153, 12.50000000000000000, -3.637306695894650055 ) ) ;
#36769=ORIENTED_EDGE ( 'NONE', *, *, #49020, .T. ) ;
#36770=VERTEX_POINT ( 'NONE', #87424 ) ;
#36771=CIRCLE ( 'NONE', #61903, 0.1000000000000002554 ) ;
#36772=VERTEX_POINT ( 'NONE', #114317 ) ;
#36773=DIRECTION ( 'NONE',  ( -0.000000000000000000, -1.000000000000000000, -0.000000000000000000 ) ) ;
#36774=AXIS2_PLACEMENT_3D ( 'NONE', #110122, #47991, #129148 ) ;
#36775=VECTOR ( 'NONE', #5461, 1000.000000000000000 ) ;
#36776=CARTESIAN_POINT ( 'NONE',  ( 13.74999999999989697, 2.500000000000000000, 2.957883832488649389 ) ) ;
#36777=CARTESIAN_POINT ( 'NONE',  ( -3.749999999999994671, 2.500000000000000000, -6.395190528383301931 ) ) ;
#36778=CIRCLE ( 'NONE', #126649, 0.1000000000000000472 ) ;
#36779=DIRECTION ( 'NONE',  ( 0.000000000000000000, 1.000000000000000000, 0.000000000000000000 ) ) ;
#36780=DIRECTION ( 'NONE',  ( -0.000000000000000000, 1.000000000000000000, -0.000000000000000000 ) ) ;
#36781=CARTESIAN_POINT ( 'NONE',  ( 9.999999999999911182, 12.50000000000000000, -3.637306695894650055 ) ) ;
#36782=ORIENTED_EDGE ( 'NONE', *, *, #113737, .T. ) ;
#36783=DIRECTION ( 'NONE',  ( 0.000000000000000000, 1.000000000000000000, 0.000000000000000000 ) ) ;
#36784=ORIENTED_EDGE ( 'NONE', *, *, #39977, .F. ) ;
#36785=AXIS2_PLACEMENT_3D ( 'NONE', #63415, #84340, #122347 ) ;
#36786=VERTEX_POINT ( 'NONE', #24654 ) ;
#36787=ORIENTED_EDGE ( 'NONE', *, *, #43414, .T. ) ;
#36788=ADVANCED_FACE ( 'NONE', ( #37699 ), #36501, .T. ) ;
#36789=ORIENTED_EDGE ( 'NONE', *, *, #91351, .F. ) ;
#36790=CIRCLE ( 'NONE', #34739, 0.06509327318403745899 ) ;
#36791=CARTESIAN_POINT ( 'NONE',  ( -7.900000000000014566, 12.50000000000000000, -2.276824562219559311E-15 ) ) ;
#36792=VERTEX_POINT ( 'NONE', #20644 ) ;
#36793=ORIENTED_EDGE ( 'NONE', *, *, #34539, .T. ) ;
#36794=ADVANCED_FACE ( 'NONE', ( #9525 ), #72090, .T. ) ;
#36795=AXIS2_PLACEMENT_3D ( 'NONE', #60246, #18358, #39948 ) ;
#36796=CARTESIAN_POINT ( 'NONE',  ( 4.199999999999941558, 12.50000000000000000, -4.330127018922201643 ) ) ;
#36797=DIRECTION ( 'NONE',  ( 0.000000000000000000, 0.000000000000000000, 1.000000000000000000 ) ) ;
#36798=CARTESIAN_POINT ( 'NONE',  ( -9.150000000000009237, 2.500000000000000000, -1.372243186433550033 ) ) ;
#36799=DIRECTION ( 'NONE',  ( 0.000000000000000000, 0.000000000000000000, 1.000000000000000000 ) ) ;
#36800=ORIENTED_EDGE ( 'NONE', *, *, #33082, .F. ) ;
#36801=CARTESIAN_POINT ( 'NONE',  ( 7.099999999999926814, 12.50000000000000000, -0.6928203230275541413 ) ) ;
#36802=ORIENTED_EDGE ( 'NONE', *, *, #78593, .F. ) ;
#36803=LINE ( 'NONE', #96335, #31725 ) ;
#36804=ORIENTED_EDGE ( 'NONE', *, *, #34101, .F. ) ;
#36805=LINE ( 'NONE', #127749, #113156 ) ;
#36806=EDGE_LOOP ( 'NONE', ( #3578, #86017, #108697, #31705 ) ) ;
#36807=ORIENTED_EDGE ( 'NONE', *, *, #110312, .F. ) ;
#36808=CARTESIAN_POINT ( 'NONE',  ( -4.150000000000024336, 12.50000000000000000, 2.165063509461097713 ) ) ;
#36809=DIRECTION ( 'NONE',  ( 0.000000000000000000, -0.000000000000000000, 1.000000000000000000 ) ) ;
#36810=CIRCLE ( 'NONE', #109965, 0.1000000000000000472 ) ;
#36811=CARTESIAN_POINT ( 'NONE',  ( 11.64999999999990443, 12.50000000000000000, -5.737276932171712751 ) ) ;
#36812=AXIS2_PLACEMENT_3D ( 'NONE', #60335, #82543, #100247 ) ;
#36813=DIRECTION ( 'NONE',  ( 0.000000000000000000, -0.000000000000000000, 1.000000000000000000 ) ) ;
#36814=CARTESIAN_POINT ( 'NONE',  ( 21.24754738303276724, -0.7337760880902383098, -4.182111650399352953 ) ) ;
#36817=DIRECTION ( 'NONE',  ( -0.000000000000000000, -1.000000000000000000, -0.000000000000000000 ) ) ;
#36818=LINE ( 'NONE', #76729, #82806 ) ;
#36819=CARTESIAN_POINT ( 'NONE',  ( -10.84999999999999964, 2.500000000000000000, 5.902370205355745192 ) ) ;
#36820=CARTESIAN_POINT ( 'NONE',  ( -3.550000000000031797, 12.50000000000000000, -6.148780366869526226 ) ) ;
#36821=AXIS2_PLACEMENT_3D ( 'NONE', #17530, #57479, #18178 ) ;
#36822=DIRECTION ( 'NONE',  ( -4.274815082592931898E-19, -0.9999939076577903929, -0.003490651415223739937 ) ) ;
#36823=ADVANCED_FACE ( 'NONE', ( #29180 ), #101331, .T. ) ;
#36824=ORIENTED_EDGE ( 'NONE', *, *, #97425, .T. ) ;
#36825=ORIENTED_EDGE ( 'NONE', *, *, #95348, .T. ) ;
#36826=FACE_OUTER_BOUND ( 'NONE', #76767, .T. ) ;
#36827=ORIENTED_EDGE ( 'NONE', *, *, #35690, .T. ) ;
#36828=AXIS2_PLACEMENT_3D ( 'NONE', #97010, #55800, #87818 ) ;
#36829=DIRECTION ( 'NONE',  ( -0.000000000000000000, 1.000000000000000000, -0.000000000000000000 ) ) ;
#36830=CARTESIAN_POINT ( 'NONE',  ( -6.050000000000020250, 2.500000000000000000, -2.511473670974877948 ) ) ;
#36831=ADVANCED_FACE ( 'NONE', ( #10778 ), #51161, .T. ) ;
#36832=EDGE_CURVE ( 'NONE', #93842, #18830, #107588, .T. ) ;
#36833=ORIENTED_EDGE ( 'NONE', *, *, #26084, .F. ) ;
#36835=DIRECTION ( 'NONE',  ( 0.000000000000000000, -0.9999939076577903929, 0.003490651415223739937 ) ) ;
#36836=CARTESIAN_POINT ( 'NONE',  ( -6.249999999999984901, 2.500000000000000000, -6.495190528383302464 ) ) ;
#36837=CARTESIAN_POINT ( 'NONE',  ( -1.650000000000035660, 2.500000000000000000, 2.757883832488649656 ) ) ;
#36838=EDGE_CURVE ( 'NONE', #39278, #111575, #18037, .T. ) ;
#36839=CARTESIAN_POINT ( 'NONE',  ( -1.850000000000033396, 2.500000000000000000, -6.148780366869526226 ) ) ;
#36840=ORIENTED_EDGE ( 'NONE', *, *, #4456, .F. ) ;
#36841=CARTESIAN_POINT ( 'NONE',  ( -10.65000000000000391, 2.500000000000000000, -6.841600689897075149 ) ) ;
#36842=DIRECTION ( 'NONE',  ( 0.000000000000000000, -0.9999939076577903929, 0.003490651415223739937 ) ) ;
#36843=ADVANCED_FACE ( 'NONE', ( #8855 ), #57988, .T. ) ;
#36844=ORIENTED_EDGE ( 'NONE', *, *, #84750, .F. ) ;
#36845=EDGE_CURVE ( 'NONE', #50744, #79454, #32399, .T. ) ;
#36847=AXIS2_PLACEMENT_3D ( 'NONE', #52838, #81647, #92774 ) ;
#36848=CARTESIAN_POINT ( 'NONE',  ( -1.650000000000035660, 2.500000000000000000, 2.857883832488649301 ) ) ;
#36849=DIRECTION ( 'NONE',  ( 0.000000000000000000, 0.000000000000000000, 1.000000000000000000 ) ) ;
#36850=ORIENTED_EDGE ( 'NONE', *, *, #74047, .F. ) ;
#36851=VECTOR ( 'NONE', #88278, 1000.000000000000000 ) ;
#36852=CARTESIAN_POINT ( 'NONE',  ( 9.349999999999919709, 2.500000000000000000, 2.511473670974873507 ) ) ;
#36853=CIRCLE ( 'NONE', #120468, 0.1000000000000002554 ) ;
#36855=DIRECTION ( 'NONE',  ( 0.000000000000000000, 1.000000000000000000, 0.000000000000000000 ) ) ;
#36856=DIRECTION ( 'NONE',  ( -0.000000000000000000, -1.000000000000000000, -0.000000000000000000 ) ) ;
#36857=CARTESIAN_POINT ( 'NONE',  ( 13.09999999999990195, 2.500000000000000000, -4.676537180435978769 ) ) ;
#36858=CIRCLE ( 'NONE', #34810, 0.1000000000000002554 ) ;
#36859=ORIENTED_EDGE ( 'NONE', *, *, #66676, .F. ) ;
#36860=CARTESIAN_POINT ( 'NONE',  ( -7.300000000000014921, 2.500000000000000000, 4.676537180435972552 ) ) ;
#36861=AXIS2_PLACEMENT_3D ( 'NONE', #16238, #56175, #96107 ) ;
#36863=EDGE_LOOP ( 'NONE', ( #74409, #120241 ) ) ;
#36864=EDGE_LOOP ( 'NONE', ( #44972, #17199 ) ) ;
#36865=DIRECTION ( 'NONE',  ( 0.000000000000000000, 0.000000000000000000, 1.000000000000000000 ) ) ;
#36866=CIRCLE ( 'NONE', #78647, 0.06509327318403741736 ) ;
#36867=CIRCLE ( 'NONE', #34831, 0.06509327318403745899 ) ;
#36868=CONICAL_SURFACE ( 'NONE', #110032, 0.1000000000000002554, 0.003490658503988666988 ) ;
#36869=VERTEX_POINT ( 'NONE', #118828 ) ;
#36870=DIRECTION ( 'NONE',  ( 0.000000000000000000, 0.000000000000000000, 1.000000000000000000 ) ) ;
#36871=DIRECTION ( 'NONE',  ( 0.000000000000000000, 0.000000000000000000, -1.000000000000000000 ) ) ;
#36872=ORIENTED_EDGE ( 'NONE', *, *, #62137, .F. ) ;
#36873=ORIENTED_EDGE ( 'NONE', *, *, #73166, .T. ) ;
#36874=DIRECTION ( 'NONE',  ( 0.000000000000000000, 1.000000000000000000, 0.000000000000000000 ) ) ;
#36875=DIRECTION ( 'NONE',  ( -0.000000000000000000, 1.000000000000000000, -0.000000000000000000 ) ) ;
#36876=ORIENTED_EDGE ( 'NONE', *, *, #64156, .F. ) ;
#36877=EDGE_CURVE ( 'NONE', #49835, #32336, #122263, .T. ) ;
#36878=CARTESIAN_POINT ( 'NONE',  ( 13.14999999999990088, 2.500000000000000000, 2.611473670974873151 ) ) ;
#36879=DIRECTION ( 'NONE',  ( -4.274815082592931898E-19, -0.9999939076577903929, -0.003490651415223739937 ) ) ;
#36880=CARTESIAN_POINT ( 'NONE',  ( -3.750000000000026201, 2.500000000000000000, 5.902370205355745192 ) ) ;
#36881=DIRECTION ( 'NONE',  ( 0.000000000000000000, -0.9999939076577903929, 0.003490651415223739937 ) ) ;
#36882=ADVANCED_FACE ( 'NONE', ( #48817 ), #1058, .T. ) ;
#36883=CARTESIAN_POINT ( 'NONE',  ( 1.849999999999948130, 2.500000000000000000, 6.148780366869520009 ) ) ;
#36884=DIRECTION ( 'NONE',  ( -0.000000000000000000, 1.000000000000000000, -0.000000000000000000 ) ) ;
#36885=EDGE_CURVE ( 'NONE', #118223, #67418, #38351, .T. ) ;
#36886=EDGE_CURVE ( 'NONE', #3107, #75929, #108360, .T. ) ;
#36887=ORIENTED_EDGE ( 'NONE', *, *, #58968, .T. ) ;
#36888=VERTEX_POINT ( 'NONE', #50735 ) ;
#36889=EDGE_CURVE ( 'NONE', #34079, #29998, #107675, .T. ) ;
#36890=ORIENTED_EDGE ( 'NONE', *, *, #8523, .F. ) ;
#36891=EDGE_LOOP ( 'NONE', ( #113849, #79687 ) ) ;
#36892=DIRECTION ( 'NONE',  ( 0.000000000000000000, 0.000000000000000000, 1.000000000000000000 ) ) ;
#36893=CARTESIAN_POINT ( 'NONE',  ( -6.050000000000018474, 12.50000000000000000, 6.841600689897072485 ) ) ;
#36894=CARTESIAN_POINT ( 'NONE',  ( -7.900000000000014566, 2.500000000000000000, -0.7928203230275542301 ) ) ;
#36895=ORIENTED_EDGE ( 'NONE', *, *, #77345, .F. ) ;
#36896=FACE_BOUND ( 'NONE', #38851, .T. ) ;
#36897=FACE_OUTER_BOUND ( 'NONE', #16738, .T. ) ;
#36898=DIRECTION ( 'NONE',  ( 0.000000000000000000, 1.000000000000000000, 0.000000000000000000 ) ) ;
#36899=EDGE_CURVE ( 'NONE', #45123, #117938, #124403, .T. ) ;
#36900=PLANE ( 'NONE',  #43016 ) ;
#36901=EDGE_CURVE ( 'NONE', #44118, #3657, #65898, .T. ) ;
#36902=VECTOR ( 'NONE', #24836, 1000.000000000000000 ) ;
#36903=PLANE ( 'NONE',  #99296 ) ;
#36904=VECTOR ( 'NONE', #32662, 1000.000000000000000 ) ;
#36905=DIRECTION ( 'NONE',  ( 0.000000000000000000, 0.000000000000000000, -1.000000000000000000 ) ) ;
#36906=DIRECTION ( 'NONE',  ( -0.000000000000000000, 1.000000000000000000, -0.000000000000000000 ) ) ;
#36907=DIRECTION ( 'NONE',  ( 0.000000000000000000, 0.000000000000000000, -1.000000000000000000 ) ) ;
#36908=LINE ( 'NONE', #108205, #84779 ) ;
#36909=FACE_OUTER_BOUND ( 'NONE', #118563, .T. ) ;
#36910=DIRECTION ( 'NONE',  ( 0.000000000000000000, 1.000000000000000000, 0.000000000000000000 ) ) ;
#36911=AXIS2_PLACEMENT_3D ( 'NONE', #109431, #11218, #79966 ) ;
#36912=AXIS2_PLACEMENT_3D ( 'NONE', #59095, #98351, #75649 ) ;
#36913=ORIENTED_EDGE ( 'NONE', *, *, #13769, .F. ) ;
#36914=ORIENTED_EDGE ( 'NONE', *, *, #87975, .F. ) ;
#36915=EDGE_LOOP ( 'NONE', ( #127961, #93799, #73848, #71347 ) ) ;
#36916=EDGE_LOOP ( 'NONE', ( #14662, #37841 ) ) ;
#36917=CARTESIAN_POINT ( 'NONE',  ( 17.48307833624011209, -2.102402844586175323, -4.293715869774332283 ) ) ;
#36918=DIRECTION ( 'NONE',  ( 0.000000000000000000, 0.000000000000000000, 1.000000000000000000 ) ) ;
#36920=ORIENTED_EDGE ( 'NONE', *, *, #23266, .F. ) ;
#36921=VERTEX_POINT ( 'NONE', #99849 ) ;
#36922=LINE ( 'NONE', #106922, #10279 ) ;
#36923=AXIS2_PLACEMENT_3D ( 'NONE', #118574, #119229, #110689 ) ;
#36924=AXIS2_PLACEMENT_3D ( 'NONE', #120566, #70814, #5919 ) ;
#36925=AXIS2_PLACEMENT_3D ( 'NONE', #3282, #24854, #123058 ) ;
#36926=CARTESIAN_POINT ( 'NONE',  ( 6.714630671503883264, -2.499999999999365397, 9.763603585388606731 ) ) ;
#36927=CARTESIAN_POINT ( 'NONE',  ( 11.24999999999990763, 2.500000000000000000, -7.188010851410854052 ) ) ;
#36928=CARTESIAN_POINT ( 'NONE',  ( -8.550000000000007816, 2.500000000000000000, 6.148780366869520009 ) ) ;
#36929=CARTESIAN_POINT ( 'NONE',  ( 0.5999999999999555689, 12.50000000000000000, 4.676537180435972552 ) ) ;
#36930=ORIENTED_EDGE ( 'NONE', *, *, #79877, .F. ) ;
#36931=ORIENTED_EDGE ( 'NONE', *, *, #83144, .T. ) ;
#36932=ORIENTED_EDGE ( 'NONE', *, *, #64013, .T. ) ;
#36933=ORIENTED_EDGE ( 'NONE', *, *, #79862, .T. ) ;
#36934=DIRECTION ( 'NONE',  ( 0.000000000000000000, 0.000000000000000000, 1.000000000000000000 ) ) ;
#36935=ORIENTED_EDGE ( 'NONE', *, *, #95915, .T. ) ;
#36936=AXIS2_PLACEMENT_3D ( 'NONE', #78455, #58164, #47692 ) ;
#36937=ORIENTED_EDGE ( 'NONE', *, *, #38473, .T. ) ;
#36938=AXIS2_PLACEMENT_3D ( 'NONE', #34343, #55884, #84706 ) ;
#36939=DIRECTION ( 'NONE',  ( -4.274815082592931898E-19, -0.9999939076577903929, -0.003490651415223739937 ) ) ;
#36940=ADVANCED_FACE ( 'NONE', ( #10172 ), #119459, .T. ) ;
#36941=CARTESIAN_POINT ( 'NONE',  ( -11.44999999999999751, 2.500000000000000000, 2.611473670974873151 ) ) ;
#36942=LINE ( 'NONE', #25826, #91761 ) ;
#36943=AXIS2_PLACEMENT_3D ( 'NONE', #68388, #30430, #29134 ) ;
#36944=DIRECTION ( 'NONE',  ( 0.000000000000000000, 0.000000000000000000, 1.000000000000000000 ) ) ;
#36945=FACE_OUTER_BOUND ( 'NONE', #12601, .T. ) ;
#36946=CIRCLE ( 'NONE', #108029, 0.06509327318403745899 ) ;
#36947=ORIENTED_EDGE ( 'NONE', *, *, #29468, .F. ) ;
#36948=CARTESIAN_POINT ( 'NONE',  ( 9.349999999999916156, 12.50000000000000000, -1.818653347947326138 ) ) ;
#36949=AXIS2_PLACEMENT_3D ( 'NONE', #75341, #67261, #38515 ) ;
#36950=ORIENTED_EDGE ( 'NONE', *, *, #93458, .T. ) ;
#36951=AXIS2_PLACEMENT_3D ( 'NONE', #81881, #60967, #112014 ) ;
#36952=CARTESIAN_POINT ( 'NONE',  ( 6.849999999999929479, 2.500000000000000000, -1.818653347947326138 ) ) ;
#36953=VERTEX_POINT ( 'NONE', #50112 ) ;
#36955=DIRECTION ( 'NONE',  ( 0.000000000000000000, 1.000000000000000000, 0.000000000000000000 ) ) ;
#36956=EDGE_LOOP ( 'NONE', ( #55595, #6218 ) ) ;
#36957=CARTESIAN_POINT ( 'NONE',  ( -2.900000000000029221, 2.500000000000000000, -5.022947341949754119 ) ) ;
#36958=CONICAL_SURFACE ( 'NONE', #110103, 0.09999999999999982514, 0.003490658503988666988 ) ;
#36959=DIRECTION ( 'NONE',  ( -0.000000000000000000, -1.000000000000000000, -0.000000000000000000 ) ) ;
#36960=EDGE_LOOP ( 'NONE', ( #39028, #125873, #6625, #105908 ) ) ;
#36961=AXIS2_PLACEMENT_3D ( 'NONE', #84664, #115382, #93843 ) ;
#36962=AXIS2_PLACEMENT_3D ( 'NONE', #1026, #1660, #40977 ) ;
#36963=AXIS2_PLACEMENT_3D ( 'NONE', #28201, #77937, #71178 ) ;
#36964=DIRECTION ( 'NONE',  ( 0.000000000000000000, 1.000000000000000000, 0.000000000000000000 ) ) ;
#36965=VERTEX_POINT ( 'NONE', #89999 ) ;
#36966=ORIENTED_EDGE ( 'NONE', *, *, #95769, .T. ) ;
#36967=CARTESIAN_POINT ( 'NONE',  ( 13.34999999999989662, 12.50000000000000000, -2.857883832488653741 ) ) ;
#36968=CARTESIAN_POINT ( 'NONE',  ( -2.300000000000032685, 2.500000000000000000, -0.3464101615137783474 ) ) ;
#36970=CARTESIAN_POINT ( 'NONE',  ( 11.84999999999990727, 2.500000000000000000, -1.918653347947326004 ) ) ;
#36971=CARTESIAN_POINT ( 'NONE',  ( 2.899999999999945732, 12.50000000000000000, -4.330127018922201643 ) ) ;
#36972=DIRECTION ( 'NONE',  ( 0.000000000000000000, 1.000000000000000000, 0.000000000000000000 ) ) ;
#36973=AXIS2_PLACEMENT_3D ( 'NONE', #5014, #15479, #63954 ) ;
#36974=ORIENTED_EDGE ( 'NONE', *, *, #52279, .F. ) ;
#36975=DIRECTION ( 'NONE',  ( 0.000000000000000000, 0.000000000000000000, 1.000000000000000000 ) ) ;
#36976=EDGE_CURVE ( 'NONE', #109372, #71330, #51266, .T. ) ;
#36977=ORIENTED_EDGE ( 'NONE', *, *, #68458, .F. ) ;
#36978=EDGE_CURVE ( 'NONE', #64891, #224, #82130, .T. ) ;
#36979=PLANE ( 'NONE',  #37103 ) ;
#36980=CARTESIAN_POINT ( 'NONE',  ( 10.64999999999991331, 2.500000000000000000, -2.411473670974877859 ) ) ;
#36981=DIRECTION ( 'NONE',  ( -0.000000000000000000, -1.000000000000000000, -0.000000000000000000 ) ) ;
#36982=DIRECTION ( 'NONE',  ( -0.000000000000000000, -1.000000000000000000, -0.000000000000000000 ) ) ;
#36983=EDGE_CURVE ( 'NONE', #27754, #74400, #57503, .T. ) ;
#36984=DIRECTION ( 'NONE',  ( 0.000000000000000000, 1.000000000000000000, 0.000000000000000000 ) ) ;
#36985=ORIENTED_EDGE ( 'NONE', *, *, #10221, .F. ) ;
#36986=CIRCLE ( 'NONE', #3624, 0.06509327318403745899 ) ;
#36987=AXIS2_PLACEMENT_3D ( 'NONE', #9458, #70312, #49399 ) ;
#36988=DIRECTION ( 'NONE',  ( 0.000000000000000000, 1.000000000000000000, 0.000000000000000000 ) ) ;
#36989=CARTESIAN_POINT ( 'NONE',  ( 6.049999999999932321, 2.500000000000000000, -1.718653347947326049 ) ) ;
#36990=EDGE_CURVE ( 'NONE', #72747, #43219, #115987, .T. ) ;
#36991=ADVANCED_FACE ( 'NONE', ( #32419 ), #55443, .T. ) ;
#36992=ADVANCED_FACE ( 'NONE', ( #40945 ), #63790, .T. ) ;
#36993=EDGE_CURVE ( 'NONE', #118684, #102955, #5253, .T. ) ;
#36994=EDGE_LOOP ( 'NONE', ( #64081, #44697, #23454, #53946 ) ) ;
#36995=CONICAL_SURFACE ( 'NONE', #22439, 0.09999999999999982514, 0.003490658503988666988 ) ;
#36996=AXIS2_PLACEMENT_3D ( 'NONE', #61681, #101593, #22403 ) ;
#36997=CARTESIAN_POINT ( 'NONE',  ( -9.600000000000008527, 2.500000000000000000, -3.637306695894645614 ) ) ;
#36998=EDGE_LOOP ( 'NONE', ( #89988, #31729, #90378, #100131 ) ) ;
#36999=VERTEX_POINT ( 'NONE', #2936 ) ;
#37000=CARTESIAN_POINT ( 'NONE',  ( -14.14999999999998792, 12.50000000000000000, 2.857883832488652853 ) ) ;
#37001=ADVANCED_FACE ( 'NONE', ( #12724 ), #110928, .T. ) ;
#37002=VERTEX_POINT ( 'NONE', #12094 ) ;
#37003=LINE ( 'NONE', #68380, #73737 ) ;
#37004=LINE ( 'NONE', #78225, #58936 ) ;
#37005=CIRCLE ( 'NONE', #112314, 0.09999999999999982514 ) ;
#37006=VECTOR ( 'NONE', #77265, 1000.000000000000000 ) ;
#37007=CARTESIAN_POINT ( 'NONE',  ( 0.8499999999999550138, 2.500000000000000000, -5.902370205355750521 ) ) ;
#37008=ORIENTED_EDGE ( 'NONE', *, *, #5883, .F. ) ;
#37009=VECTOR ( 'NONE', #31730, 1000.000000000000000 ) ;
#37010=FACE_BOUND ( 'NONE', #94498, .T. ) ;
#37011=DIRECTION ( 'NONE',  ( 0.000000000000000000, -0.9999939076577903929, 0.003490651415223739937 ) ) ;
#37012=ORIENTED_EDGE ( 'NONE', *, *, #113142, .F. ) ;
#37013=CARTESIAN_POINT ( 'NONE',  ( 1.899999999999951283, 2.500000000000000000, -0.4464101615137782142 ) ) ;
#37014=CARTESIAN_POINT ( 'NONE',  ( -4.600000000000025402, 12.50000000000000000, -0.06509327318403980434 ) ) ;
#37015=VERTEX_POINT ( 'NONE', #42882 ) ;
#37016=ORIENTED_EDGE ( 'NONE', *, *, #39020, .T. ) ;
#37017=VERTEX_POINT ( 'NONE', #11452 ) ;
#37018=DIRECTION ( 'NONE',  ( 0.000000000000000000, -0.9999939076577903929, 0.003490651415223739937 ) ) ;
#37019=CARTESIAN_POINT ( 'NONE',  ( -5.600000000000020073, 2.500000000000000000, -0.4464101615137782142 ) ) ;
#37020=DIRECTION ( 'NONE',  ( -4.274815082592931898E-19, -0.9999939076577903929, -0.003490651415223739937 ) ) ;
#37021=EDGE_CURVE ( 'NONE', #46732, #110704, #34538, .T. ) ;
#37022=FACE_BOUND ( 'NONE', #75223, .T. ) ;
#37023=EDGE_LOOP ( 'NONE', ( #62015, #51658 ) ) ;
#37024=CONICAL_SURFACE ( 'NONE', #16062, 0.1000000000000002554, 0.003490658503988666988 ) ;
#37025=CIRCLE ( 'NONE', #114374, 0.1000000000000002554 ) ;
#37027=FACE_OUTER_BOUND ( 'NONE', #63183, .T. ) ;
#37028=AXIS2_PLACEMENT_3D ( 'NONE', #70873, #112736, #32898 ) ;
#37029=CARTESIAN_POINT ( 'NONE',  ( -9.550000000000006040, 2.500000000000000000, -2.165063509461101710 ) ) ;
#37030=VECTOR ( 'NONE', #113472, 1000.000000000000000 ) ;
#37031=CARTESIAN_POINT ( 'NONE',  ( 4.799999999999935874, 12.50000000000000000, 4.048810130592458201 ) ) ;
#37032=ADVANCED_FACE ( 'NONE', ( #91302 ), #82794, .T. ) ;
#37033=DIRECTION ( 'NONE',  ( 0.000000000000000000, 0.000000000000000000, 1.000000000000000000 ) ) ;
#37034=EDGE_CURVE ( 'NONE', #4134, #44028, #99277, .T. ) ;
#37035=DIRECTION ( 'NONE',  ( 0.000000000000000000, 0.000000000000000000, 1.000000000000000000 ) ) ;
#37036=VECTOR ( 'NONE', #51404, 1000.000000000000000 ) ;
#37037=FACE_OUTER_BOUND ( 'NONE', #128862, .T. ) ;
#37038=ADVANCED_FACE ( 'NONE', ( #41587 ), #30335, .T. ) ;
#37039=AXIS2_PLACEMENT_3D ( 'NONE', #37063, #56031, #45591 ) ;
#37040=AXIS2_PLACEMENT_3D ( 'NONE', #57102, #126497, #16516 ) ;
#37041=EDGE_CURVE ( 'NONE', #12469, #95314, #65801, .T. ) ;
#37042=VERTEX_POINT ( 'NONE', #13381 ) ;
#37043=ORIENTED_EDGE ( 'NONE', *, *, #113826, .F. ) ;
#37044=ORIENTED_EDGE ( 'NONE', *, *, #13327, .T. ) ;
#37045=ORIENTED_EDGE ( 'NONE', *, *, #95094, .T. ) ;
#37046=ORIENTED_EDGE ( 'NONE', *, *, #60683, .F. ) ;
#37047=CARTESIAN_POINT ( 'NONE',  ( -9.150000000000009237, 2.500000000000000000, 2.757883832488649656 ) ) ;
#37048=EDGE_CURVE ( 'NONE', #109438, #106434, #26110, .T. ) ;
#37049=DIRECTION ( 'NONE',  ( 0.000000000000000000, 0.000000000000000000, -1.000000000000000000 ) ) ;
#37050=VERTEX_POINT ( 'NONE', #123345 ) ;
#37051=EDGE_CURVE ( 'NONE', #82756, #16935, #126465, .T. ) ;
#37052=FACE_BOUND ( 'NONE', #89565, .T. ) ;
#37053=AXIS2_PLACEMENT_3D ( 'NONE', #89815, #40084, #108800 ) ;
#37054=CARTESIAN_POINT ( 'NONE',  ( 12.49999999999990052, 2.500000000000000000, 0.5928203230275495006 ) ) ;
#37055=EDGE_CURVE ( 'NONE', #41488, #28130, #90656, .T. ) ;
#37056=ADVANCED_FACE ( 'NONE', ( #31748 ), #103470, .T. ) ;
#37057=CIRCLE ( 'NONE', #32958, 0.06509327318403745899 ) ;
#37058=AXIS2_PLACEMENT_3D ( 'NONE', #73745, #82308, #64580 ) ;
#37059=EDGE_CURVE ( 'NONE', #121575, #88292, #59589, .T. ) ;
#37060=CARTESIAN_POINT ( 'NONE',  ( 14.99999999999992895, 12.50000000000000000, 0.06509327318403515528 ) ) ;
#37061=CARTESIAN_POINT ( 'NONE',  ( 8.949999999999917577, 12.50000000000000000, 6.148780366869520009 ) ) ;
#37062=DIRECTION ( 'NONE',  ( 0.000000000000000000, 0.000000000000000000, 1.000000000000000000 ) ) ;
#37063=CARTESIAN_POINT ( 'NONE',  ( 13.09999999999989839, 12.50000000000000000, 0.3464101615137735735 ) ) ;
#37064=EDGE_LOOP ( 'NONE', ( #74453, #16806, #628, #100582 ) ) ;
#37065=DIRECTION ( 'NONE',  ( 0.000000000000000000, 0.000000000000000000, 1.000000000000000000 ) ) ;
#37066=ADVANCED_FACE ( 'NONE', ( #54582 ), #11525, .T. ) ;
#37067=VERTEX_POINT ( 'NONE', #104967 ) ;
#37068=ORIENTED_EDGE ( 'NONE', *, *, #78517, .T. ) ;
#37069=ORIENTED_EDGE ( 'NONE', *, *, #72381, .F. ) ;
#37071=DIRECTION ( 'NONE',  ( 0.000000000000000000, 0.000000000000000000, -1.000000000000000000 ) ) ;
#37072=CARTESIAN_POINT ( 'NONE',  ( -1.050000000000037792, 2.500000000000000000, 1.818653347947321475 ) ) ;
#37073=ORIENTED_EDGE ( 'NONE', *, *, #50809, .F. ) ;
#37074=CONICAL_SURFACE ( 'NONE', #112373, 0.1000000000000002554, 0.003490658503988666988 ) ;
#37075=CARTESIAN_POINT ( 'NONE',  ( 2.499999999999981792, 2.500000000000000000, 4.330127018922196314 ) ) ;
#37076=FACE_OUTER_BOUND ( 'NONE', #39619, .T. ) ;
#37077=DIRECTION ( 'NONE',  ( -0.000000000000000000, -1.000000000000000000, -0.000000000000000000 ) ) ;
#37079=DIRECTION ( 'NONE',  ( -4.274815082592931898E-19, -0.9999939076577903929, -0.003490651415223739937 ) ) ;
#37080=PLANE ( 'NONE',  #69660 ) ;
#37081=CARTESIAN_POINT ( 'NONE',  ( -5.400000000000020783, 2.500000000000000000, 0.5928203230275495006 ) ) ;
#37082=VERTEX_POINT ( 'NONE', #44137 ) ;
#37083=DIRECTION ( 'NONE',  ( 0.000000000000000000, 1.000000000000000000, 0.000000000000000000 ) ) ;
#37084=AXIS2_PLACEMENT_3D ( 'NONE', #19867, #18569, #47394 ) ;
#37085=ORIENTED_EDGE ( 'NONE', *, *, #108031, .T. ) ;
#37087=EDGE_LOOP ( 'NONE', ( #91564, #45405 ) ) ;
#37088=CARTESIAN_POINT ( 'NONE',  ( -6.850000000000013856, 2.500000000000000000, 6.741600689897071952 ) ) ;
#37089=CARTESIAN_POINT ( 'NONE',  ( -9.150000000000009237, 2.500000000000000000, 1.472243186433545459 ) ) ;
#37090=CARTESIAN_POINT ( 'NONE',  ( 3.349999999999942801, 12.50000000000000000, 2.857883832488649301 ) ) ;
#37091=ORIENTED_EDGE ( 'NONE', *, *, #762, .T. ) ;
#37093=CIRCLE ( 'NONE', #95578, 0.06509327318403745899 ) ;
#37094=ORIENTED_EDGE ( 'NONE', *, *, #115691, .F. ) ;
#37095=DIRECTION ( 'NONE',  ( 0.000000000000000000, 0.000000000000000000, 1.000000000000000000 ) ) ;
#37096=CIRCLE ( 'NONE', #110243, 0.06509327318403741736 ) ;
#37097=EDGE_CURVE ( 'NONE', #7181, #7665, #84682, .T. ) ;
#37098=CARTESIAN_POINT ( 'NONE',  ( 26.74600275967221208, 2.978654849834052154, -2.722800557139402500 ) ) ;
#37099=DIRECTION ( 'NONE',  ( 0.000000000000000000, 1.000000000000000000, 0.000000000000000000 ) ) ;
#37100=ORIENTED_EDGE ( 'NONE', *, *, #41893, .T. ) ;
#37101=ORIENTED_EDGE ( 'NONE', *, *, #118716, .F. ) ;
#37102=CARTESIAN_POINT ( 'NONE',  ( 10.64999999999990976, 12.50000000000000000, -6.841600689897077814 ) ) ;
#37103=AXIS2_PLACEMENT_3D ( 'NONE', #76900, #106985, #17299 ) ;
#37105=ORIENTED_EDGE ( 'NONE', *, *, #47603, .F. ) ;
#37106=DIRECTION ( 'NONE',  ( -0.000000000000000000, -1.000000000000000000, -0.000000000000000000 ) ) ;
#37107=CIRCLE ( 'NONE', #53818, 0.1000000000000002554 ) ;
#37108=DIRECTION ( 'NONE',  ( 0.000000000000000000, 0.000000000000000000, 1.000000000000000000 ) ) ;
#37109=ORIENTED_EDGE ( 'NONE', *, *, #84735, .F. ) ;
#37110=CARTESIAN_POINT ( 'NONE',  ( 11.64999999999990443, 2.500000000000000000, 2.857883832488649301 ) ) ;
#37111=DIRECTION ( 'NONE',  ( 0.000000000000000000, -0.000000000000000000, 1.000000000000000000 ) ) ;
#37112=CARTESIAN_POINT ( 'NONE',  ( -7.900000000000014566, 12.50000000000000000, -0.7579135962115916003 ) ) ;
#37113=ADVANCED_FACE ( 'NONE', ( #76827 ), #32488, .T. ) ;
#37114=CARTESIAN_POINT ( 'NONE',  ( -12.04999999999999538, 2.500000000000000000, 2.165063509461097713 ) ) ;
#37115=EDGE_LOOP ( 'NONE', ( #82160, #13364, #7011, #123045 ) ) ;
#37116=CARTESIAN_POINT ( 'NONE',  ( -11.64999999999999680, 12.50000000000000000, 2.857883832488649301 ) ) ;
#37117=CIRCLE ( 'NONE', #41330, 0.06509327318403745899 ) ;
#37118=DIRECTION ( 'NONE',  ( -0.000000000000000000, 1.000000000000000000, -0.000000000000000000 ) ) ;
#37119=CIRCLE ( 'NONE', #76824, 0.09999999999999999167 ) ;
#37120=EDGE_LOOP ( 'NONE', ( #43824, #86028, #24811, #54507 ) ) ;
#37121=ORIENTED_EDGE ( 'NONE', *, *, #39273, .F. ) ;
#37123=FACE_OUTER_BOUND ( 'NONE', #37213, .T. ) ;
#37124=DIRECTION ( 'NONE',  ( -0.000000000000000000, 1.000000000000000000, -0.000000000000000000 ) ) ;
#37125=LINE ( 'NONE', #87484, #20873 ) ;
#37126=AXIS2_PLACEMENT_3D ( 'NONE', #69247, #119009, #18218 ) ;
#37127=CARTESIAN_POINT ( 'NONE',  ( -1.250000000000035749, 2.500000000000000000, -2.857883832488653741 ) ) ;
#37128=AXIS2_PLACEMENT_3D ( 'NONE', #121098, #100178, #50423 ) ;
#37129=DIRECTION ( 'NONE',  ( 0.000000000000000000, 0.000000000000000000, -1.000000000000000000 ) ) ;
#37130=AXIS2_PLACEMENT_3D ( 'NONE', #59226, #87354, #29120 ) ;
#37131=DIRECTION ( 'NONE',  ( 0.000000000000000000, 0.000000000000000000, 1.000000000000000000 ) ) ;
#37132=LINE ( 'NONE', #6335, #70002 ) ;
#37133=DIRECTION ( 'NONE',  ( 0.000000000000000000, 1.000000000000000000, 0.000000000000000000 ) ) ;
#37134=AXIS2_PLACEMENT_3D ( 'NONE', #22434, #61707, #62976 ) ;
#37135=CONICAL_SURFACE ( 'NONE', #116530, 0.1000000000000000056, 0.003490658503988666988 ) ;
#37136=CARTESIAN_POINT ( 'NONE',  ( -5.650000000000023448, 2.500000000000000000, -1.818653347947326138 ) ) ;
#37137=AXIS2_PLACEMENT_3D ( 'NONE', #10679, #29705, #119362 ) ;
#37138=CIRCLE ( 'NONE', #78910, 0.06509327318403745899 ) ;
#37139=EDGE_CURVE ( 'NONE', #37472, #118696, #106910, .T. ) ;
#37140=VERTEX_POINT ( 'NONE', #45437 ) ;
#37141=CARTESIAN_POINT ( 'NONE',  ( -7.900000000000011013, 12.50000000000000000, 3.572213422710607489 ) ) ;
#37143=DIRECTION ( 'NONE',  ( 0.000000000000000000, 0.000000000000000000, 1.000000000000000000 ) ) ;
#37144=CARTESIAN_POINT ( 'NONE',  ( 5.399999999999932854, 12.50000000000000000, 3.637306695894644726 ) ) ;
#37145=CARTESIAN_POINT ( 'NONE',  ( -3.749999999999991118, 2.500000000000000000, -2.165063509461101710 ) ) ;
#37146=ADVANCED_FACE ( 'NONE', ( #46079 ), #113937, .T. ) ;
#37147=VERTEX_POINT ( 'NONE', #74246 ) ;
#37148=CARTESIAN_POINT ( 'NONE',  ( -1.250000000000036193, 12.50000000000000000, 1.472243186433545459 ) ) ;
#37149=AXIS2_PLACEMENT_3D ( 'NONE', #67014, #57214, #118061 ) ;
#37150=AXIS2_PLACEMENT_3D ( 'NONE', #36848, #45381, #97044 ) ;
#37151=CARTESIAN_POINT ( 'NONE',  ( -6.650000000000014566, 12.50000000000000000, 6.495190528383297135 ) ) ;
#37152=CARTESIAN_POINT ( 'NONE',  ( 1.649999999999949729, 12.50000000000000000, 5.802370205355744659 ) ) ;
#37153=VERTEX_POINT ( 'NONE', #115424 ) ;
#37154=ADVANCED_FACE ( 'NONE', ( #96442 ), #109736, .T. ) ;
#37155=ADVANCED_FACE ( 'NONE', ( #53963 ), #63767, .T. ) ;
#37156=EDGE_CURVE ( 'NONE', #25512, #89644, #13570, .T. ) ;
#37157=EDGE_CURVE ( 'NONE', #112116, #121499, #122446, .T. ) ;
#37158=ADVANCED_FACE ( 'NONE', ( #6754 ), #65993, .T. ) ;
#37159=EDGE_LOOP ( 'NONE', ( #113047, #42546, #43801, #11606 ) ) ;
#37160=VERTEX_POINT ( 'NONE', #84704 ) ;
#37161=ORIENTED_EDGE ( 'NONE', *, *, #1652, .T. ) ;
#37162=ORIENTED_EDGE ( 'NONE', *, *, #11829, .T. ) ;
#37164=AXIS2_PLACEMENT_3D ( 'NONE', #98689, #100006, #108525 ) ;
#37165=EDGE_CURVE ( 'NONE', #94349, #43625, #101513, .T. ) ;
#37166=CARTESIAN_POINT ( 'NONE',  ( -9.350000000000006750, 2.500000000000000000, 2.511473670974873507 ) ) ;
#37167=DIRECTION ( 'NONE',  ( 0.000000000000000000, 0.000000000000000000, 1.000000000000000000 ) ) ;
#37168=ADVANCED_FACE ( 'NONE', ( #15944 ), #124635, .T. ) ;
#37169=LINE ( 'NONE', #48258, #8065 ) ;
#37170=EDGE_CURVE ( 'NONE', #98821, #79461, #26302, .T. ) ;
#37171=ORIENTED_EDGE ( 'NONE', *, *, #45432, .F. ) ;
#37172=DIRECTION ( 'NONE',  ( 0.000000000000000000, -0.000000000000000000, 1.000000000000000000 ) ) ;
#37173=ORIENTED_EDGE ( 'NONE', *, *, #80459, .F. ) ;
#37175=CARTESIAN_POINT ( 'NONE',  ( 14.38463633656414942, -2.499999999998971489, -7.683002074691544614 ) ) ;
#37176=DIRECTION ( 'NONE',  ( 0.000000000000000000, 0.000000000000000000, 1.000000000000000000 ) ) ;
#37177=CARTESIAN_POINT ( 'NONE',  ( 20.25366426269196296, -2.573118374675439135, 4.179292740210999391 ) ) ;
#37178=VERTEX_POINT ( 'NONE', #66977 ) ;
#37179=AXIS2_PLACEMENT_3D ( 'NONE', #114043, #33560, #73459 ) ;
#37180=AXIS2_PLACEMENT_3D ( 'NONE', #80630, #62278, #120543 ) ;
#37181=EDGE_LOOP ( 'NONE', ( #33253, #33089, #15732, #13535 ) ) ;
#37182=ORIENTED_EDGE ( 'NONE', *, *, #46082, .F. ) ;
#37183=ORIENTED_EDGE ( 'NONE', *, *, #56735, .T. ) ;
#37184=CARTESIAN_POINT ( 'NONE',  ( 1.449999999999950440, 2.500000000000000000, 6.148780366869520009 ) ) ;
#37185=CARTESIAN_POINT ( 'NONE',  ( 9.599999999999914380, 12.50000000000000000, -4.957854068765716882 ) ) ;
#37186=CARTESIAN_POINT ( 'NONE',  ( 14.59999999999989484, 2.500000000000000000, 0.09999999999999772959 ) ) ;
#37187=FACE_BOUND ( 'NONE', #79665, .T. ) ;
#37188=DIRECTION ( 'NONE',  ( 0.000000000000000000, 0.000000000000000000, 1.000000000000000000 ) ) ;
#37189=CARTESIAN_POINT ( 'NONE',  ( -12.04999999999999716, 12.50000000000000000, -6.430097255199260786 ) ) ;
#37190=AXIS2_PLACEMENT_3D ( 'NONE', #85391, #26480, #119354 ) ;
#37191=DIRECTION ( 'NONE',  ( 0.000000000000000000, 1.000000000000000000, 0.000000000000000000 ) ) ;
#37192=DIRECTION ( 'NONE',  ( 0.000000000000000000, 1.000000000000000000, 0.000000000000000000 ) ) ;
#37193=AXIS2_PLACEMENT_3D ( 'NONE', #13079, #62849, #40002 ) ;
#37195=CARTESIAN_POINT ( 'NONE',  ( -8.100000000000013856, 2.500000000000000000, -4.576537180435977348 ) ) ;
#37196=CARTESIAN_POINT ( 'NONE',  ( 9.149999999999920419, 2.500000000000000000, -5.802370205355749988 ) ) ;
#37197=CIRCLE ( 'NONE', #35151, 0.1000000000000002554 ) ;
#37198=DIRECTION ( 'NONE',  ( -0.000000000000000000, -1.000000000000000000, -0.000000000000000000 ) ) ;
#37199=EDGE_LOOP ( 'NONE', ( #91082, #105335 ) ) ;
#37200=ORIENTED_EDGE ( 'NONE', *, *, #95725, .F. ) ;
#37201=ORIENTED_EDGE ( 'NONE', *, *, #58801, .F. ) ;
#37202=VERTEX_POINT ( 'NONE', #65043 ) ;
#37203=VECTOR ( 'NONE', #89917, 1000.000000000000000 ) ;
#37204=CARTESIAN_POINT ( 'NONE',  ( -2.100000000000034728, 12.50000000000000000, 4.330127018922196314 ) ) ;
#37205=ADVANCED_FACE ( 'NONE', ( #6131 ), #114035, .T. ) ;
#37206=FACE_BOUND ( 'NONE', #127115, .T. ) ;
#37207=FACE_OUTER_BOUND ( 'NONE', #124263, .T. ) ;
#37208=DIRECTION ( 'NONE',  ( 0.000000000000000000, 0.000000000000000000, -1.000000000000000000 ) ) ;
#37209=EDGE_CURVE ( 'NONE', #100004, #47911, #36908, .T. ) ;
#37210=CIRCLE ( 'NONE', #24679, 0.06509327318403745899 ) ;
#37211=EDGE_CURVE ( 'NONE', #5343, #114031, #63855, .T. ) ;
#37212=AXIS2_PLACEMENT_3D ( 'NONE', #51269, #2787, #33555 ) ;
#37213=EDGE_LOOP ( 'NONE', ( #20581, #41023, #84398, #101804 ) ) ;
#37214=LINE ( 'NONE', #117020, #94838 ) ;
#37215=DIRECTION ( 'NONE',  ( 0.000000000000000000, 1.000000000000000000, 0.000000000000000000 ) ) ;
#37216=AXIS2_PLACEMENT_3D ( 'NONE', #37575, #77481, #27729 ) ;
#37217=ORIENTED_EDGE ( 'NONE', *, *, #96363, .T. ) ;
#37218=LINE ( 'NONE', #70370, #40770 ) ;
#37219=DIRECTION ( 'NONE',  ( -4.274815082592931898E-19, -0.9999939076577903929, -0.003490651415223739937 ) ) ;
#37220=ADVANCED_FACE ( 'NONE', ( #118669 ), #19945, .T. ) ;
#37221=CIRCLE ( 'NONE', #81134, 0.06509327318403745899 ) ;
#37222=VERTEX_POINT ( 'NONE', #8697 ) ;
#37223=FACE_OUTER_BOUND ( 'NONE', #1715, .T. ) ;
#37224=CARTESIAN_POINT ( 'NONE',  ( 2.049999999999950084, 2.500000000000000000, -6.395190528383301931 ) ) ;
#37225=CIRCLE ( 'NONE', #37134, 0.06509327318403743123 ) ;
#37226=CONICAL_SURFACE ( 'NONE', #120552, 0.1000000000000002554, 0.003490658503988666988 ) ;
#37227=EDGE_LOOP ( 'NONE', ( #1174, #9227, #86246, #3573 ) ) ;
#37229=CARTESIAN_POINT ( 'NONE',  ( 3.749999999999975131, 12.50000000000000000, 6.495190528383297135 ) ) ;
#37230=DIRECTION ( 'NONE',  ( -0.000000000000000000, 1.000000000000000000, -0.000000000000000000 ) ) ;
#37231=VERTEX_POINT ( 'NONE', #119310 ) ;
#37232=FACE_OUTER_BOUND ( 'NONE', #54123, .T. ) ;
#37233=ORIENTED_EDGE ( 'NONE', *, *, #65640, .F. ) ;
#37234=VERTEX_POINT ( 'NONE', #27707 ) ;
#37235=CIRCLE ( 'NONE', #89539, 0.06509327318403741736 ) ;
#37236=DIRECTION ( 'NONE',  ( -0.000000000000000000, 1.000000000000000000, -0.000000000000000000 ) ) ;
#37237=EDGE_CURVE ( 'NONE', #89246, #6208, #18540, .T. ) ;
#37238=ORIENTED_EDGE ( 'NONE', *, *, #126161, .F. ) ;
#37239=CARTESIAN_POINT ( 'NONE',  ( 1.249999999999953815, 2.500000000000000000, 1.372243186433545370 ) ) ;
#37240=FACE_BOUND ( 'NONE', #26648, .T. ) ;
#37241=CIRCLE ( 'NONE', #108319, 0.06509327318403745899 ) ;
#37242=CIRCLE ( 'NONE', #53958, 0.09999999999999999167 ) ;
#37243=ORIENTED_EDGE ( 'NONE', *, *, #85171, .T. ) ;
#37244=DIRECTION ( 'NONE',  ( 0.000000000000000000, 1.000000000000000000, 0.000000000000000000 ) ) ;
#37246=CARTESIAN_POINT ( 'NONE',  ( -8.350000000000012079, 2.500000000000000000, -1.472243186433550122 ) ) ;
#37248=DIRECTION ( 'NONE',  ( 0.000000000000000000, 0.000000000000000000, 1.000000000000000000 ) ) ;
#37249=CARTESIAN_POINT ( 'NONE',  ( 10.79999999999991012, 2.500000000000000000, 4.330127018922196314 ) ) ;
#37250=CARTESIAN_POINT ( 'NONE',  ( -8.950000000000009948, 12.50000000000000000, -1.753560074763288679 ) ) ;
#37251=EDGE_LOOP ( 'NONE', ( #78207, #95643, #13803, #20650 ) ) ;
#37252=VERTEX_POINT ( 'NONE', #19163 ) ;
#37253=FACE_OUTER_BOUND ( 'NONE', #48923, .T. ) ;
#37254=EDGE_CURVE ( 'NONE', #109616, #119283, #7395, .T. ) ;
#37255=CARTESIAN_POINT ( 'NONE',  ( 20.80940928220343267, -0.7000174339600890860, 4.161255421338324822 ) ) ;
#37256=DIRECTION ( 'NONE',  ( -0.000000000000000000, -1.000000000000000000, -0.000000000000000000 ) ) ;
#37258=EDGE_LOOP ( 'NONE', ( #14392, #103133 ) ) ;
#37259=ORIENTED_EDGE ( 'NONE', *, *, #69519, .F. ) ;
#37260=CARTESIAN_POINT ( 'NONE',  ( -12.69999999999999041, 12.50000000000000000, 4.048810130592458201 ) ) ;
#37261=CARTESIAN_POINT ( 'NONE',  ( -0.6500000000000389910, 12.50000000000000000, -1.753560074763288679 ) ) ;
#37262=CARTESIAN_POINT ( 'NONE',  ( -7.300000000000016698, 2.500000000000000000, -4.676537180435978769 ) ) ;
#37263=DIRECTION ( 'NONE',  ( 0.000000000000000000, -0.9999939076577903929, 0.003490651415223739937 ) ) ;
#37264=CARTESIAN_POINT ( 'NONE',  ( -6.450000000000014388, 2.500000000000000000, 6.048780366869521252 ) ) ;
#37265=CIRCLE ( 'NONE', #53977, 0.09999999999999982514 ) ;
#37266=AXIS2_PLACEMENT_3D ( 'NONE', #114505, #115127, #86984 ) ;
#37267=CARTESIAN_POINT ( 'NONE',  ( -3.750000000000027534, 12.50000000000000000, -1.537336459617587581 ) ) ;
#37268=DIRECTION ( 'NONE',  ( 0.000000000000000000, 0.000000000000000000, 1.000000000000000000 ) ) ;
#37269=DIRECTION ( 'NONE',  ( 0.000000000000000000, -0.000000000000000000, 1.000000000000000000 ) ) ;
#37270=AXIS2_PLACEMENT_3D ( 'NONE', #58156, #9026, #48984 ) ;
#37271=ADVANCED_FACE ( 'NONE', ( #59124 ), #82650, .T. ) ;
#37272=DIRECTION ( 'NONE',  ( 0.000000000000000000, 1.000000000000000000, 0.000000000000000000 ) ) ;
#37273=CONICAL_SURFACE ( 'NONE', #120784, 0.1000000000000002554, 0.003490658503988666988 ) ;
#37274=VERTEX_POINT ( 'NONE', #39505 ) ;
#37275=CIRCLE ( 'NONE', #83337, 0.1000000000000000472 ) ;
#37276=CARTESIAN_POINT ( 'NONE',  ( -15.39999999999997904, 12.50000000000000000, -0.6928203230275519209 ) ) ;
#37277=EDGE_LOOP ( 'NONE', ( #3210, #43076 ) ) ;
#37278=ORIENTED_EDGE ( 'NONE', *, *, #59161, .F. ) ;
#37279=CARTESIAN_POINT ( 'NONE',  ( 11.64999999999990266, 12.50000000000000000, -6.560283801567339701 ) ) ;
#37280=DIRECTION ( 'NONE',  ( 0.000000000000000000, 1.000000000000000000, 0.000000000000000000 ) ) ;
#37281=CARTESIAN_POINT ( 'NONE',  ( 13.29999999999990301, 2.500000000000000000, 4.430127018922196847 ) ) ;
#37282=CIRCLE ( 'NONE', #129327, 0.1000000000000002554 ) ;
#37283=PLANE ( 'NONE',  #25359 ) ;
#37284=VECTOR ( 'NONE', #102676, 1000.000000000000000 ) ;
#37285=DIRECTION ( 'NONE',  ( 0.000000000000000000, 1.000000000000000000, 0.000000000000000000 ) ) ;
#37286=DIRECTION ( 'NONE',  ( -4.274815082592931898E-19, -0.9999939076577903929, -0.003490651415223739937 ) ) ;
#37287=CARTESIAN_POINT ( 'NONE',  ( 5.649999999999932854, 2.500000000000000000, 1.918653347947321564 ) ) ;
#37288=ORIENTED_EDGE ( 'NONE', *, *, #123583, .F. ) ;
#37289=DIRECTION ( 'NONE',  ( 0.000000000000000000, 0.000000000000000000, 1.000000000000000000 ) ) ;
#37290=DIRECTION ( 'NONE',  ( 0.000000000000000000, 1.000000000000000000, 0.000000000000000000 ) ) ;
#37291=AXIS2_PLACEMENT_3D ( 'NONE', #96762, #48324, #88215 ) ;
#37292=ORIENTED_EDGE ( 'NONE', *, *, #110057, .T. ) ;
#37293=EDGE_CURVE ( 'NONE', #77665, #48600, #72276, .T. ) ;
#37294=VERTEX_POINT ( 'NONE', #67628 ) ;
#37295=ORIENTED_EDGE ( 'NONE', *, *, #50425, .F. ) ;
#37296=ORIENTED_EDGE ( 'NONE', *, *, #110254, .T. ) ;
#37297=CARTESIAN_POINT ( 'NONE',  ( 6.249999999999932498, 12.50000000000000000, -5.802370205355749988 ) ) ;
#37298=CARTESIAN_POINT ( 'NONE',  ( -10.40000000000000213, 2.500000000000000000, -2.276824562219559311E-15 ) ) ;
#37299=EDGE_CURVE ( 'NONE', #100004, #118058, #78543, .T. ) ;
#37300=CIRCLE ( 'NONE', #3835, 0.06509327318403745899 ) ;
#37301=ORIENTED_EDGE ( 'NONE', *, *, #80337, .F. ) ;
#37302=DIRECTION ( 'NONE',  ( 0.000000000000000000, 1.000000000000000000, 0.000000000000000000 ) ) ;
#37303=CARTESIAN_POINT ( 'NONE',  ( 2.500000000000002220, 2.750000000000000000, -9.999999999999998224 ) ) ;
#37305=CARTESIAN_POINT ( 'NONE',  ( 2.299999999999946976, 2.500000000000000000, 4.676537180435972552 ) ) ;
#37306=EDGE_LOOP ( 'NONE', ( #25296, #74863, #29032, #12026 ) ) ;
#37307=ADVANCED_FACE ( 'NONE', ( #37553 ), #48019, .T. ) ;
#37308=EDGE_CURVE ( 'NONE', #67061, #128241, #47365, .T. ) ;
#37309=EDGE_CURVE ( 'NONE', #93927, #65479, #80586, .T. ) ;
#37310=CARTESIAN_POINT ( 'NONE',  ( 9.599999999999914380, 12.50000000000000000, 5.022947341949748790 ) ) ;
#37311=EDGE_CURVE ( 'NONE', #108239, #55973, #86828, .T. ) ;
#37312=AXIS2_PLACEMENT_3D ( 'NONE', #2967, #84085, #93923 ) ;
#37313=DIRECTION ( 'NONE',  ( 0.000000000000000000, 1.000000000000000000, 0.000000000000000000 ) ) ;
#37314=ORIENTED_EDGE ( 'NONE', *, *, #29185, .F. ) ;
#37315=CIRCLE ( 'NONE', #89528, 0.1000000000000000472 ) ;
#37316=VERTEX_POINT ( 'NONE', #87904 ) ;
#37317=ADVANCED_FACE ( 'NONE', ( #59788 ), #5352, .T. ) ;
#37318=ORIENTED_EDGE ( 'NONE', *, *, #42184, .F. ) ;
#37319=DIRECTION ( 'NONE',  ( 0.000000000000000000, 0.000000000000000000, 1.000000000000000000 ) ) ;
#37320=EDGE_CURVE ( 'NONE', #125752, #10577, #17869, .T. ) ;
#37322=ADVANCED_FACE ( 'NONE', ( #68277 ), #93225, .T. ) ;
#37323=CARTESIAN_POINT ( 'NONE',  ( -6.450000000000019718, 2.500000000000000000, -6.248780366869526759 ) ) ;
#37324=ADVANCED_FACE ( 'NONE', ( #12697 ), #123316, .T. ) ;
#37325=EDGE_CURVE ( 'NONE', #30816, #26142, #34629, .T. ) ;
#37327=FACE_OUTER_BOUND ( 'NONE', #20868, .T. ) ;
#37328=DIRECTION ( 'NONE',  ( 0.000000000000000000, 0.000000000000000000, 1.000000000000000000 ) ) ;
#37330=DIRECTION ( 'NONE',  ( 0.000000000000000000, 0.000000000000000000, 1.000000000000000000 ) ) ;
#37332=EDGE_CURVE ( 'NONE', #112983, #64387, #99367, .T. ) ;
#37333=VERTEX_POINT ( 'NONE', #114145 ) ;
#37334=AXIS2_PLACEMENT_3D ( 'NONE', #6968, #65912, #105845 ) ;
#37335=CARTESIAN_POINT ( 'NONE',  ( 0.3999999999999559464, 12.50000000000000000, -4.330127018922201643 ) ) ;
#37336=VERTEX_POINT ( 'NONE', #121377 ) ;
#37337=VERTEX_POINT ( 'NONE', #43485 ) ;
#37338=CARTESIAN_POINT ( 'NONE',  ( -3.350000000000028955, 12.50000000000000000, -2.099970236277064473 ) ) ;
#37339=VERTEX_POINT ( 'NONE', #63104 ) ;
#37340=CARTESIAN_POINT ( 'NONE',  ( -1.650000000000035216, 2.500000000000000000, -5.702370205355749455 ) ) ;
#37341=FACE_BOUND ( 'NONE', #105654, .T. ) ;
#37342=DIRECTION ( 'NONE',  ( 0.000000000000000000, 1.000000000000000000, 0.000000000000000000 ) ) ;
#37343=DIRECTION ( 'NONE',  ( -0.000000000000000000, -1.000000000000000000, -0.000000000000000000 ) ) ;
#37344=DIRECTION ( 'NONE',  ( 0.000000000000000000, 1.000000000000000000, 0.000000000000000000 ) ) ;
#37345=VERTEX_POINT ( 'NONE', #81470 ) ;
#37346=CARTESIAN_POINT ( 'NONE',  ( 4.149999999999939959, 12.50000000000000000, 1.472243186433545459 ) ) ;
#37347=LINE ( 'NONE', #85774, #2938 ) ;
#37348=DIRECTION ( 'NONE',  ( 0.000000000000000000, 0.000000000000000000, 1.000000000000000000 ) ) ;
#37349=DIRECTION ( 'NONE',  ( 0.000000000000000000, 0.000000000000000000, 1.000000000000000000 ) ) ;
#37350=ORIENTED_EDGE ( 'NONE', *, *, #54697, .F. ) ;
#37351=DIRECTION ( 'NONE',  ( 0.000000000000000000, 0.000000000000000000, -1.000000000000000000 ) ) ;
#37352=AXIS2_PLACEMENT_3D ( 'NONE', #53075, #22341, #43274 ) ;
#37353=AXIS2_PLACEMENT_3D ( 'NONE', #5541, #36959, #85404 ) ;
#37354=DIRECTION ( 'NONE',  ( 0.000000000000000000, 0.000000000000000000, 1.000000000000000000 ) ) ;
#37355=CIRCLE ( 'NONE', #29045, 0.06509327318403745899 ) ;
#37356=ORIENTED_EDGE ( 'NONE', *, *, #43113, .T. ) ;
#37357=DIRECTION ( 'NONE',  ( -0.000000000000000000, 1.000000000000000000, -0.000000000000000000 ) ) ;
#37358=CARTESIAN_POINT ( 'NONE',  ( 13.34999999999989662, 2.500000000000000000, -1.472243186433550122 ) ) ;
#37359=FACE_BOUND ( 'NONE', #101452, .T. ) ;
#37360=CARTESIAN_POINT ( 'NONE',  ( -6.450000000000017941, 12.50000000000000000, -6.841600689897077814 ) ) ;
#37361=CIRCLE ( 'NONE', #49888, 0.1000000000000000472 ) ;
#37362=CONICAL_SURFACE ( 'NONE', #120873, 0.1000000000000002554, 0.003490658503988666988 ) ;
#37363=EDGE_CURVE ( 'NONE', #6764, #44454, #68047, .T. ) ;
#37364=CIRCLE ( 'NONE', #87507, 0.06509327318403743123 ) ;
#37365=ORIENTED_EDGE ( 'NONE', *, *, #46632, .F. ) ;
#37366=DIRECTION ( 'NONE',  ( -0.000000000000000000, 1.000000000000000000, -0.000000000000000000 ) ) ;
#37367=CIRCLE ( 'NONE', #116763, 0.06509327318403745899 ) ;
#37368=EDGE_CURVE ( 'NONE', #120641, #37017, #1599, .T. ) ;
#37369=VERTEX_POINT ( 'NONE', #122671 ) ;
#37370=VERTEX_POINT ( 'NONE', #31720 ) ;
#37371=CARTESIAN_POINT ( 'NONE',  ( -9.800000000000007816, 2.500000000000000000, -3.883716857408422207 ) ) ;
#37373=ORIENTED_EDGE ( 'NONE', *, *, #83082, .T. ) ;
#37374=CARTESIAN_POINT ( 'NONE',  ( -11.84999999999999787, 2.500000000000000000, -6.048780366869523029 ) ) ;
#37375=FACE_OUTER_BOUND ( 'NONE', #93716, .T. ) ;
#37377=AXIS2_PLACEMENT_3D ( 'NONE', #24889, #65445, #16958 ) ;
#37379=CONICAL_SURFACE ( 'NONE', #5949, 0.1000000000000000472, 0.003490658503988666988 ) ;
#37380=EDGE_LOOP ( 'NONE', ( #25089, #100801 ) ) ;
#37381=CARTESIAN_POINT ( 'NONE',  ( -1.650000000000035216, 2.500000000000000000, -1.472243186433550122 ) ) ;
#37382=DIRECTION ( 'NONE',  ( -0.000000000000000000, -1.000000000000000000, -0.000000000000000000 ) ) ;
#37383=PLANE ( 'NONE',  #103564 ) ;
#37384=VECTOR ( 'NONE', #60332, 1000.000000000000000 ) ;
#37385=CARTESIAN_POINT ( 'NONE',  ( 18.45986577996938394, 0.7763546025154585140, -4.045836809868015749 ) ) ;
#37386=EDGE_LOOP ( 'NONE', ( #39535, #76966 ) ) ;
#37387=CARTESIAN_POINT ( 'NONE',  ( 6.899999999999928413, 2.500000000000000000, -3.983716857408426293 ) ) ;
#37388=ORIENTED_EDGE ( 'NONE', *, *, #32195, .T. ) ;
#37389=CARTESIAN_POINT ( 'NONE',  ( 2.099999999999950351, 2.500000000000000000, -2.276824562219559311E-15 ) ) ;
#37390=CARTESIAN_POINT ( 'NONE',  ( 6.049999999999935874, 2.500000000000000000, -6.841600689897077814 ) ) ;
#37391=ORIENTED_EDGE ( 'NONE', *, *, #8610, .F. ) ;
#37392=DIRECTION ( 'NONE',  ( 0.000000000000000000, 1.000000000000000000, 0.000000000000000000 ) ) ;
#37393=CARTESIAN_POINT ( 'NONE',  ( -0.8500000000000382805, 2.500000000000000000, -2.957883832488653830 ) ) ;
#37394=FACE_OUTER_BOUND ( 'NONE', #32247, .T. ) ;
#37395=LINE ( 'NONE', #36756, #73760 ) ;
#37396=ORIENTED_EDGE ( 'NONE', *, *, #64334, .F. ) ;
#37397=AXIS2_PLACEMENT_3D ( 'NONE', #118893, #78340, #387 ) ;
#37398=DIRECTION ( 'NONE',  ( 0.000000000000000000, 0.000000000000000000, 1.000000000000000000 ) ) ;
#37399=LINE ( 'NONE', #77308, #33456 ) ;
#37401=DIRECTION ( 'NONE',  ( 0.000000000000000000, -0.000000000000000000, 1.000000000000000000 ) ) ;
#37402=AXIS2_PLACEMENT_3D ( 'NONE', #27745, #76864, #36308 ) ;
#37403=CARTESIAN_POINT ( 'NONE',  ( 10.19999999999991047, 2.500000000000000000, 4.676537180435972552 ) ) ;
#37404=EDGE_CURVE ( 'NONE', #4260, #124496, #95253, .T. ) ;
#37405=ORIENTED_EDGE ( 'NONE', *, *, #5369, .F. ) ;
#37406=VERTEX_POINT ( 'NONE', #113492 ) ;
#37407=DIRECTION ( 'NONE',  ( 0.000000000000000000, 1.000000000000000000, 0.000000000000000000 ) ) ;
#37408=ORIENTED_EDGE ( 'NONE', *, *, #88906, .T. ) ;
#37409=CARTESIAN_POINT ( 'NONE',  ( -0.6500000000000394351, 12.50000000000000000, 2.446380397790835826 ) ) ;
#37410=ORIENTED_EDGE ( 'NONE', *, *, #62660, .T. ) ;
#37411=EDGE_LOOP ( 'NONE', ( #68690, #63111 ) ) ;
#37412=ORIENTED_EDGE ( 'NONE', *, *, #96284, .F. ) ;
#37413=CIRCLE ( 'NONE', #10212, 0.1000000000000002554 ) ;
#37414=DIRECTION ( 'NONE',  ( 0.000000000000000000, 0.000000000000000000, 1.000000000000000000 ) ) ;
#37415=DIRECTION ( 'NONE',  ( 0.000000000000000000, 1.000000000000000000, 0.000000000000000000 ) ) ;
#37416=DIRECTION ( 'NONE',  ( -4.274815082592931898E-19, -0.9999939076577903929, -0.003490651415223739937 ) ) ;
#37418=CONICAL_SURFACE ( 'NONE', #24884, 0.09999999999999982514, 0.003490658503988666988 ) ;
#37419=CIRCLE ( 'NONE', #10218, 0.09999999999999982514 ) ;
#37420=DIRECTION ( 'NONE',  ( 0.000000000000000000, 1.000000000000000000, 0.000000000000000000 ) ) ;
#37421=CARTESIAN_POINT ( 'NONE',  ( -0.4500000000000397571, 2.500000000000000000, -6.395190528383301931 ) ) ;
#37422=EDGE_CURVE ( 'NONE', #80982, #95427, #25526, .T. ) ;
#37423=DIRECTION ( 'NONE',  ( 0.000000000000000000, 1.000000000000000000, 0.000000000000000000 ) ) ;
#37424=AXIS2_PLACEMENT_3D ( 'NONE', #33816, #52813, #84848 ) ;
#37425=ORIENTED_EDGE ( 'NONE', *, *, #99457, .F. ) ;
#37426=EDGE_CURVE ( 'NONE', #96763, #58128, #91928, .T. ) ;
#37427=CARTESIAN_POINT ( 'NONE',  ( -4.400000000000025224, 2.500000000000000000, 4.676537180435972552 ) ) ;
#37428=EDGE_LOOP ( 'NONE', ( #45654, #83977, #127279, #73984 ) ) ;
#37429=CIRCLE ( 'NONE', #125239, 0.06509327318403745899 ) ;
#37430=AXIS2_PLACEMENT_3D ( 'NONE', #24603, #92045, #43613 ) ;
#37431=EDGE_LOOP ( 'NONE', ( #78878, #96183 ) ) ;
#37432=ORIENTED_EDGE ( 'NONE', *, *, #74389, .T. ) ;
#37433=ORIENTED_EDGE ( 'NONE', *, *, #1864, .F. ) ;
#37434=DIRECTION ( 'NONE',  ( 0.000000000000000000, 0.000000000000000000, 1.000000000000000000 ) ) ;
#37435=ORIENTED_EDGE ( 'NONE', *, *, #81302, .F. ) ;
#37436=ADVANCED_FACE ( 'NONE', ( #14627 ), #36679, .T. ) ;
#37437=VERTEX_POINT ( 'NONE', #83406 ) ;
#37438=CARTESIAN_POINT ( 'NONE',  ( -8.300000000000011369, 12.50000000000000000, -4.330127018922201643 ) ) ;
#37439=CARTESIAN_POINT ( 'NONE',  ( 8.299999999999922551, 2.500000000000000000, -2.385244779468109755E-15 ) ) ;
#37440=CARTESIAN_POINT ( 'NONE',  ( 1.449999999999952216, 2.500000000000000000, 1.718653347947321386 ) ) ;
#37441=CARTESIAN_POINT ( 'NONE',  ( -5.400000000000023448, 12.50000000000000000, -5.022947341949754119 ) ) ;
#37442=DIRECTION ( 'NONE',  ( 0.000000000000000000, 0.000000000000000000, 1.000000000000000000 ) ) ;
#37443=CIRCLE ( 'NONE', #81355, 0.06509327318403745899 ) ;
#37444=ORIENTED_EDGE ( 'NONE', *, *, #46024, .F. ) ;
#37445=LINE ( 'NONE', #118558, #42916 ) ;
#37446=ORIENTED_EDGE ( 'NONE', *, *, #16403, .T. ) ;
#37447=FACE_OUTER_BOUND ( 'NONE', #8900, .T. ) ;
#37448=AXIS2_PLACEMENT_3D ( 'NONE', #12319, #21506, #52258 ) ;
#37449=EDGE_LOOP ( 'NONE', ( #102369, #126192, #67548, #89589 ) ) ;
#37450=CARTESIAN_POINT ( 'NONE',  ( -7.500000000000015099, 2.500000000000000000, -0.5928203230275541635 ) ) ;
#37451=ORIENTED_EDGE ( 'NONE', *, *, #37311, .T. ) ;
#37452=ORIENTED_EDGE ( 'NONE', *, *, #14793, .F. ) ;
#37453=DIRECTION ( 'NONE',  ( 0.000000000000000000, 0.000000000000000000, 1.000000000000000000 ) ) ;
#37454=CIRCLE ( 'NONE', #54174, 0.06509327318403745899 ) ;
#37455=CARTESIAN_POINT ( 'NONE',  ( 1.899999999999951283, 2.500000000000000000, -3.983716857408426293 ) ) ;
#37456=AXIS2_PLACEMENT_3D ( 'NONE', #71222, #121602, #31962 ) ;
#37457=EDGE_CURVE ( 'NONE', #87251, #12173, #76380, .T. ) ;
#37458=AXIS2_PLACEMENT_3D ( 'NONE', #129034, #100811, #79274 ) ;
#37459=CARTESIAN_POINT ( 'NONE',  ( 13.09999999999989839, 12.50000000000000000, -0.3464101615137783474 ) ) ;
#37460=CARTESIAN_POINT ( 'NONE',  ( -9.400000000000007461, 2.500000000000000000, 3.883716857408420431 ) ) ;
#37462=EDGE_LOOP ( 'NONE', ( #17355, #33113, #85266, #9434 ) ) ;
#37463=CARTESIAN_POINT ( 'NONE',  ( -12.89999999999999147, 12.50000000000000000, -4.395220292106237103 ) ) ;
#37464=FACE_OUTER_BOUND ( 'NONE', #28018, .T. ) ;
#37465=ADVANCED_FACE ( 'NONE', ( #52011 ), #63762, .T. ) ;
#37467=DIRECTION ( 'NONE',  ( 0.000000000000000000, 0.000000000000000000, 1.000000000000000000 ) ) ;
#37468=CIRCLE ( 'NONE', #14440, 0.06509327318403745899 ) ;
#37469=ADVANCED_FACE ( 'NONE', ( #53937 ), #30426, .T. ) ;
#37470=DIRECTION ( 'NONE',  ( 0.000000000000000000, 0.000000000000000000, 1.000000000000000000 ) ) ;
#37471=AXIS2_PLACEMENT_3D ( 'NONE', #90895, #102009, #33289 ) ;
#37472=VERTEX_POINT ( 'NONE', #82106 ) ;
#37473=ORIENTED_EDGE ( 'NONE', *, *, #34227, .F. ) ;
#37474=EDGE_CURVE ( 'NONE', #93025, #118854, #13663, .T. ) ;
#37475=EDGE_CURVE ( 'NONE', #32318, #46996, #116184, .T. ) ;
#37476=DIRECTION ( 'NONE',  ( 0.000000000000000000, 0.000000000000000000, -1.000000000000000000 ) ) ;
#37477=ADVANCED_FACE ( 'NONE', ( #104943 ), #55857, .T. ) ;
#37478=VERTEX_POINT ( 'NONE', #35593 ) ;
#37479=DIRECTION ( 'NONE',  ( 0.000000000000000000, 0.000000000000000000, 1.000000000000000000 ) ) ;
#37480=CARTESIAN_POINT ( 'NONE',  ( 6.249999999999932498, 2.500000000000000000, -2.857883832488653741 ) ) ;
#37481=EDGE_CURVE ( 'NONE', #97670, #48086, #45175, .T. ) ;
#37482=CIRCLE ( 'NONE', #110616, 0.06509327318403745899 ) ;
#37483=VERTEX_POINT ( 'NONE', #26417 ) ;
#37485=DIRECTION ( 'NONE',  ( -0.000000000000000000, 1.000000000000000000, -0.000000000000000000 ) ) ;
#37486=EDGE_CURVE ( 'NONE', #59157, #64666, #55627, .T. ) ;
#37487=CARTESIAN_POINT ( 'NONE',  ( 8.949999999999917577, 12.50000000000000000, 6.148780366869520009 ) ) ;
#37488=CARTESIAN_POINT ( 'NONE',  ( 0.1999999999999576006, 2.500000000000000000, -4.576537180435978236 ) ) ;
#37489=EDGE_LOOP ( 'NONE', ( #112764, #15012 ) ) ;
#37490=EDGE_CURVE ( 'NONE', #114315, #47981, #80677, .T. ) ;
#37491=DIRECTION ( 'NONE',  ( 0.000000000000000000, 0.000000000000000000, -1.000000000000000000 ) ) ;
#37492=DIRECTION ( 'NONE',  ( 0.000000000000000000, 0.000000000000000000, 1.000000000000000000 ) ) ;
#37493=EDGE_LOOP ( 'NONE', ( #88497, #111785, #37665, #18291 ) ) ;
#37494=FACE_OUTER_BOUND ( 'NONE', #127774, .T. ) ;
#37495=AXIS2_PLACEMENT_3D ( 'NONE', #125163, #17772, #106792 ) ;
#37496=LINE ( 'NONE', #56461, #12089 ) ;
#37497=DIRECTION ( 'NONE',  ( 0.000000000000000000, 1.000000000000000000, 0.000000000000000000 ) ) ;
#37498=EDGE_LOOP ( 'NONE', ( #21065, #45007 ) ) ;
#37499=DIRECTION ( 'NONE',  ( 0.000000000000000000, 0.000000000000000000, 1.000000000000000000 ) ) ;
#37500=ORIENTED_EDGE ( 'NONE', *, *, #60957, .T. ) ;
#37501=DIRECTION ( 'NONE',  ( -0.000000000000000000, -1.000000000000000000, -0.000000000000000000 ) ) ;
#37502=CIRCLE ( 'NONE', #91872, 0.06509327318403745899 ) ;
#37503=DIRECTION ( 'NONE',  ( -0.000000000000000000, -1.000000000000000000, -0.000000000000000000 ) ) ;
#37504=DIRECTION ( 'NONE',  ( 0.000000000000000000, 1.000000000000000000, 0.000000000000000000 ) ) ;
#37505=EDGE_LOOP ( 'NONE', ( #94672, #16477, #115830, #30143 ) ) ;
#37506=FACE_OUTER_BOUND ( 'NONE', #17984, .T. ) ;
#37507=AXIS2_PLACEMENT_3D ( 'NONE', #42292, #52116, #111679 ) ;
#37508=AXIS2_PLACEMENT_3D ( 'NONE', #61334, #120886, #1110 ) ;
#37509=DIRECTION ( 'NONE',  ( 0.000000000000000000, 1.000000000000000000, 0.000000000000000000 ) ) ;
#37510=VECTOR ( 'NONE', #69072, 1000.000000000000000 ) ;
#37511=EDGE_LOOP ( 'NONE', ( #97140, #29606, #74802, #112475 ) ) ;
#37512=DIRECTION ( 'NONE',  ( -0.000000000000000000, 1.000000000000000000, -0.000000000000000000 ) ) ;
#37513=ORIENTED_EDGE ( 'NONE', *, *, #59205, .F. ) ;
#37514=DIRECTION ( 'NONE',  ( 0.000000000000000000, 0.000000000000000000, 1.000000000000000000 ) ) ;
#37516=ADVANCED_FACE ( 'NONE', ( #106255 ), #16560, .T. ) ;
#37517=VERTEX_POINT ( 'NONE', #87242 ) ;
#37518=CARTESIAN_POINT ( 'NONE',  ( 6.849999999999929479, 2.500000000000000000, 6.741600689897071952 ) ) ;
#37519=DIRECTION ( 'NONE',  ( 0.000000000000000000, -0.000000000000000000, 1.000000000000000000 ) ) ;
#37520=VERTEX_POINT ( 'NONE', #96414 ) ;
#37521=ORIENTED_EDGE ( 'NONE', *, *, #101108, .T. ) ;
#37522=CARTESIAN_POINT ( 'NONE',  ( -3.100000000000028511, 2.500000000000000000, 0.2464101615137736789 ) ) ;
#37523=CARTESIAN_POINT ( 'NONE',  ( 6.249999999999932498, 2.500000000000000000, 5.802370205355744659 ) ) ;
#37524=VERTEX_POINT ( 'NONE', #27053 ) ;
#37525=EDGE_CURVE ( 'NONE', #87160, #42019, #97386, .T. ) ;
#37526=CARTESIAN_POINT ( 'NONE',  ( 10.59999999999990905, 2.500000000000000000, 4.676537180435972552 ) ) ;
#37527=DIRECTION ( 'NONE',  ( 0.000000000000000000, 1.000000000000000000, 0.000000000000000000 ) ) ;
#37528=DIRECTION ( 'NONE',  ( 0.000000000000000000, 0.000000000000000000, 1.000000000000000000 ) ) ;
#37529=CIRCLE ( 'NONE', #66751, 0.06509327318403745899 ) ;
#37531=LINE ( 'NONE', #117326, #97485 ) ;
#37532=DIRECTION ( 'NONE',  ( 0.000000000000000000, 0.000000000000000000, 1.000000000000000000 ) ) ;
#37533=CONICAL_SURFACE ( 'NONE', #121145, 0.09999999999999982514, 0.003490658503988666988 ) ;
#37534=VERTEX_POINT ( 'NONE', #126547 ) ;
#37535=ORIENTED_EDGE ( 'NONE', *, *, #87920, .T. ) ;
#37536=EDGE_LOOP ( 'NONE', ( #15351, #25226 ) ) ;
#37537=ORIENTED_EDGE ( 'NONE', *, *, #118139, .T. ) ;
#37538=CARTESIAN_POINT ( 'NONE',  ( -11.24999999999999822, 12.50000000000000000, 5.802370205355744659 ) ) ;
#37539=CARTESIAN_POINT ( 'NONE',  ( 10.44999999999991402, 2.500000000000000000, 6.495190528383297135 ) ) ;
#37540=CARTESIAN_POINT ( 'NONE',  ( 11.64999999999990621, 12.50000000000000000, -2.165063509461101710 ) ) ;
#37541=ORIENTED_EDGE ( 'NONE', *, *, #23124, .T. ) ;
#37542=FACE_BOUND ( 'NONE', #93904, .T. ) ;
#37543=CARTESIAN_POINT ( 'NONE',  ( -13.74999999999998934, 12.50000000000000000, -1.407149913249510442 ) ) ;
#37544=CARTESIAN_POINT ( 'NONE',  ( -6.900000000000019007, 2.500000000000000000, -0.4464101615137783252 ) ) ;
#37545=AXIS2_PLACEMENT_3D ( 'NONE', #24413, #22503, #52580 ) ;
#37546=AXIS2_PLACEMENT_3D ( 'NONE', #63985, #103914, #94090 ) ;
#37547=DIRECTION ( 'NONE',  ( 0.000000000000000000, 0.000000000000000000, 1.000000000000000000 ) ) ;
#37548=AXIS2_PLACEMENT_3D ( 'NONE', #85046, #115799, #74592 ) ;
#37549=DIRECTION ( 'NONE',  ( -0.000000000000000000, 1.000000000000000000, -0.000000000000000000 ) ) ;
#37550=CARTESIAN_POINT ( 'NONE',  ( -6.450000000000017941, 12.50000000000000000, -6.906693963081115051 ) ) ;
#37551=DIRECTION ( 'NONE',  ( 0.000000000000000000, 1.000000000000000000, 0.000000000000000000 ) ) ;
#37552=DIRECTION ( 'NONE',  ( 0.000000000000000000, 1.000000000000000000, 0.000000000000000000 ) ) ;
#37553=FACE_OUTER_BOUND ( 'NONE', #101909, .T. ) ;
#37554=CARTESIAN_POINT ( 'NONE',  ( -5.450000000000019718, 12.50000000000000000, 2.230156782645134950 ) ) ;
#37555=AXIS2_PLACEMENT_3D ( 'NONE', #76790, #116697, #27044 ) ;
#37556=DIRECTION ( 'NONE',  ( -0.000000000000000000, 1.000000000000000000, -0.000000000000000000 ) ) ;
#37557=AXIS2_PLACEMENT_3D ( 'NONE', #93482, #110226, #48737 ) ;
#37558=EDGE_CURVE ( 'NONE', #83877, #31984, #82833, .T. ) ;
#37559=VERTEX_POINT ( 'NONE', #36880 ) ;
#37560=ORIENTED_EDGE ( 'NONE', *, *, #6194, .T. ) ;
#37561=CIRCLE ( 'NONE', #41774, 0.06509327318403743123 ) ;
#37562=ORIENTED_EDGE ( 'NONE', *, *, #118709, .T. ) ;
#37563=ORIENTED_EDGE ( 'NONE', *, *, #14376, .T. ) ;
#37564=DIRECTION ( 'NONE',  ( 0.000000000000000000, 0.000000000000000000, 1.000000000000000000 ) ) ;
#37565=CARTESIAN_POINT ( 'NONE',  ( 1.899999999999951283, 2.500000000000000000, -4.676537180435977881 ) ) ;
#37566=ORIENTED_EDGE ( 'NONE', *, *, #111682, .T. ) ;
#37567=ORIENTED_EDGE ( 'NONE', *, *, #47656, .F. ) ;
#37568=VERTEX_POINT ( 'NONE', #116708 ) ;
#37569=LINE ( 'NONE', #77476, #54198 ) ;
#37570=ADVANCED_FACE ( 'NONE', ( #66952 ), #116158, .T. ) ;
#37571=DIRECTION ( 'NONE',  ( 0.000000000000000000, -0.000000000000000000, 1.000000000000000000 ) ) ;
#37572=FACE_OUTER_BOUND ( 'NONE', #98687, .T. ) ;
#37573=DIRECTION ( 'NONE',  ( 0.000000000000000000, -0.9999939076577903929, 0.003490651415223739937 ) ) ;
#37574=VECTOR ( 'NONE', #40804, 1000.000000000000000 ) ;
#37575=CARTESIAN_POINT ( 'NONE',  ( -3.150000000000030553, 12.50000000000000000, 6.148780366869520009 ) ) ;
#37576=EDGE_CURVE ( 'NONE', #26610, #111368, #97080, .T. ) ;
#37577=DIRECTION ( 'NONE',  ( -0.000000000000000000, -1.000000000000000000, -0.000000000000000000 ) ) ;
#37578=ADVANCED_FACE ( 'NONE', ( #4813 ), #3306, .T. ) ;
#37579=EDGE_LOOP ( 'NONE', ( #40184, #34771, #26481, #96648 ) ) ;
#37580=FACE_OUTER_BOUND ( 'NONE', #44056, .T. ) ;
#37581=ORIENTED_EDGE ( 'NONE', *, *, #118428, .F. ) ;
#37582=ORIENTED_EDGE ( 'NONE', *, *, #124943, .F. ) ;
#37583=ORIENTED_EDGE ( 'NONE', *, *, #80617, .F. ) ;
#37584=ADVANCED_FACE ( 'NONE', ( #34958 ), #76472, .T. ) ;
#37585=CARTESIAN_POINT ( 'NONE',  ( 6.849999999999927702, 12.50000000000000000, 2.511473670974873507 ) ) ;
#37587=EDGE_LOOP ( 'NONE', ( #103542, #96904 ) ) ;
#37588=ADVANCED_FACE ( 'NONE', ( #65013 ), #5438, .T. ) ;
#37589=ORIENTED_EDGE ( 'NONE', *, *, #39262, .T. ) ;
#37590=FACE_OUTER_BOUND ( 'NONE', #1818, .T. ) ;
#37591=DIRECTION ( 'NONE',  ( 0.000000000000000000, 0.000000000000000000, -1.000000000000000000 ) ) ;
#37592=CARTESIAN_POINT ( 'NONE',  ( 10.64999999999990976, 12.50000000000000000, -6.148780366869526226 ) ) ;
#37593=CARTESIAN_POINT ( 'NONE',  ( 10.44999999999991047, 2.500000000000000000, 2.165063509461097713 ) ) ;
#37594=DIRECTION ( 'NONE',  ( 0.000000000000000000, 1.000000000000000000, 0.000000000000000000 ) ) ;
#37595=CIRCLE ( 'NONE', #46001, 0.1000000000000000472 ) ;
#37596=ORIENTED_EDGE ( 'NONE', *, *, #63257, .F. ) ;
#37597=DIRECTION ( 'NONE',  ( -0.000000000000000000, 1.000000000000000000, -0.000000000000000000 ) ) ;
#37598=ORIENTED_EDGE ( 'NONE', *, *, #8608, .F. ) ;
#37599=CARTESIAN_POINT ( 'NONE',  ( 2.699999999999947331, 12.50000000000000000, -4.741630453620016006 ) ) ;
#37600=AXIS2_PLACEMENT_3D ( 'NONE', #14098, #64499, #34423 ) ;
#37601=CONICAL_SURFACE ( 'NONE', #83568, 0.1000000000000002554, 0.003490658503988666988 ) ;
#37602=ORIENTED_EDGE ( 'NONE', *, *, #57130, .F. ) ;
#37603=DIRECTION ( 'NONE',  ( -0.000000000000000000, 1.000000000000000000, -0.000000000000000000 ) ) ;
#37604=CARTESIAN_POINT ( 'NONE',  ( 21.24754738303276724, -0.7337760880902383098, -4.182111650399352953 ) ) ;
#37605=ORIENTED_EDGE ( 'NONE', *, *, #123327, .F. ) ;
#37606=CIRCLE ( 'NONE', #129561, 0.06509327318403745899 ) ;
#37607=CARTESIAN_POINT ( 'NONE',  ( -1.250000000000037970, 2.500000000000000000, 2.857883832488649301 ) ) ;
#37608=CARTESIAN_POINT ( 'NONE',  ( -11.64999999999999680, 2.500000000000000000, -2.065063509461098068 ) ) ;
#37609=ORIENTED_EDGE ( 'NONE', *, *, #73892, .F. ) ;
#37610=CIRCLE ( 'NONE', #48073, 0.1000000000000000472 ) ;
#37611=AXIS2_PLACEMENT_3D ( 'NONE', #21713, #61642, #101561 ) ;
#37612=ADVANCED_FACE ( 'NONE', ( #5459 ), #70205, .T. ) ;
#37613=CARTESIAN_POINT ( 'NONE',  ( 9.399999999999915090, 2.500000000000000000, -3.883716857408426648 ) ) ;
#37614=ORIENTED_EDGE ( 'NONE', *, *, #45039, .F. ) ;
#37615=ORIENTED_EDGE ( 'NONE', *, *, #47813, .F. ) ;
#37616=DIRECTION ( 'NONE',  ( 0.000000000000000000, 1.000000000000000000, 0.000000000000000000 ) ) ;
#37617=DIRECTION ( 'NONE',  ( 0.000000000000000000, 0.000000000000000000, 1.000000000000000000 ) ) ;
#37618=EDGE_CURVE ( 'NONE', #88926, #110204, #105804, .T. ) ;
#37620=FACE_OUTER_BOUND ( 'NONE', #43495, .T. ) ;
#37621=EDGE_CURVE ( 'NONE', #121105, #59532, #13751, .T. ) ;
#37622=CARTESIAN_POINT ( 'NONE',  ( -10.40000000000000213, 12.50000000000000000, -4.330127018922197202 ) ) ;
#37623=PLANE ( 'NONE',  #655 ) ;
#37624=EDGE_CURVE ( 'NONE', #104601, #102213, #59764, .T. ) ;
#37625=ADVANCED_FACE ( 'NONE', ( #58459 ), #51443, .T. ) ;
#37626=EDGE_CURVE ( 'NONE', #103846, #38154, #91130, .T. ) ;
#37627=ORIENTED_EDGE ( 'NONE', *, *, #29196, .F. ) ;
#37628=CARTESIAN_POINT ( 'NONE',  ( -4.550000000000026468, 12.50000000000000000, -6.560283801567339701 ) ) ;
#37629=AXIS2_PLACEMENT_3D ( 'NONE', #53256, #32350, #82728 ) ;
#37630=FACE_OUTER_BOUND ( 'NONE', #15160, .T. ) ;
#37631=CIRCLE ( 'NONE', #96185, 0.1000000000000002554 ) ;
#37632=VERTEX_POINT ( 'NONE', #147 ) ;
#37633=EDGE_CURVE ( 'NONE', #51388, #17427, #107854, .T. ) ;
#37634=CARTESIAN_POINT ( 'NONE',  ( -14.99999999999994671, 2.500000000000000000, 0.000000000000000000 ) ) ;
#37635=PLANE ( 'NONE',  #5031 ) ;
#37636=CARTESIAN_POINT ( 'NONE',  ( 11.04999999999991012, 12.50000000000000000, -1.818653347947326138 ) ) ;
#37637=DIRECTION ( 'NONE',  ( -0.000000000000000000, -1.000000000000000000, -0.000000000000000000 ) ) ;
#37638=CARTESIAN_POINT ( 'NONE',  ( -15.39999999999997904, 12.50000000000000000, -0.6928203230275519209 ) ) ;
#37639=ORIENTED_EDGE ( 'NONE', *, *, #60099, .F. ) ;
#37640=AXIS2_PLACEMENT_3D ( 'NONE', #11157, #51111, #89091 ) ;
#37641=ADVANCED_FACE ( 'NONE', ( #70840 ), #126645, .T. ) ;
#37642=EDGE_CURVE ( 'NONE', #44029, #14513, #128501, .T. ) ;
#37643=CARTESIAN_POINT ( 'NONE',  ( 2.049999999999950084, 2.500000000000000000, -2.165063509461101710 ) ) ;
#37644=VECTOR ( 'NONE', #86439, 1000.000000000000000 ) ;
#37645=ORIENTED_EDGE ( 'NONE', *, *, #9624, .F. ) ;
#37646=CARTESIAN_POINT ( 'NONE',  ( 3.949999999999941558, 12.50000000000000000, -6.213873640053564351 ) ) ;
#37647=AXIS2_PLACEMENT_3D ( 'NONE', #80620, #79961, #40047 ) ;
#37648=EDGE_LOOP ( 'NONE', ( #54342, #1454, #43438, #29340 ) ) ;
#37650=ORIENTED_EDGE ( 'NONE', *, *, #79157, .F. ) ;
#37651=DIRECTION ( 'NONE',  ( -0.000000000000000000, -1.000000000000000000, -0.000000000000000000 ) ) ;
#37652=CONICAL_SURFACE ( 'NONE', #77358, 0.1000000000000000472, 0.003490658503988666988 ) ;
#37653=ORIENTED_EDGE ( 'NONE', *, *, #102157, .F. ) ;
#37654=LINE ( 'NONE', #36372, #82064 ) ;
#37655=CARTESIAN_POINT ( 'NONE',  ( 8.749999999999920064, 12.50000000000000000, -2.857883832488653741 ) ) ;
#37656=CIRCLE ( 'NONE', #22984, 0.06509327318403745899 ) ;
#37657=DIRECTION ( 'NONE',  ( -4.274815082592931898E-19, -0.9999939076577903929, -0.003490651415223739937 ) ) ;
#37658=VERTEX_POINT ( 'NONE', #99668 ) ;
#37659=FACE_BOUND ( 'NONE', #1520, .T. ) ;
#37660=LINE ( 'NONE', #19276, #51518 ) ;
#37661=ORIENTED_EDGE ( 'NONE', *, *, #106115, .T. ) ;
#37662=CIRCLE ( 'NONE', #52318, 0.06509327318403741736 ) ;
#37663=CARTESIAN_POINT ( 'NONE',  ( -11.24999999999999822, 2.500000000000000000, 1.572243186433545548 ) ) ;
#37664=DIRECTION ( 'NONE',  ( 0.000000000000000000, 1.000000000000000000, 0.000000000000000000 ) ) ;
#37665=ORIENTED_EDGE ( 'NONE', *, *, #82669, .T. ) ;
#37668=EDGE_LOOP ( 'NONE', ( #5463, #56220, #14950, #97158 ) ) ;
#37669=CARTESIAN_POINT ( 'NONE',  ( 0.3999999999999559464, 2.500000000000000000, -4.330127018922201643 ) ) ;
#37670=DIRECTION ( 'NONE',  ( 0.000000000000000000, 0.000000000000000000, 1.000000000000000000 ) ) ;
#37671=CARTESIAN_POINT ( 'NONE',  ( -6.050000000000020250, 2.500000000000000000, -6.741600689897078169 ) ) ;
#37672=FACE_BOUND ( 'NONE', #91917, .T. ) ;
#37673=ORIENTED_EDGE ( 'NONE', *, *, #126112, .T. ) ;
#37674=DIRECTION ( 'NONE',  ( -0.000000000000000000, -1.000000000000000000, -0.000000000000000000 ) ) ;
#37675=CARTESIAN_POINT ( 'NONE',  ( 0.1999999999999567124, 12.50000000000000000, -3.983716857408426293 ) ) ;
#37676=ORIENTED_EDGE ( 'NONE', *, *, #110636, .T. ) ;
#37677=ADVANCED_FACE ( 'NONE', ( #92403 ), #86917, .T. ) ;
#37678=DIRECTION ( 'NONE',  ( 0.000000000000000000, 0.000000000000000000, 1.000000000000000000 ) ) ;
#37679=CIRCLE ( 'NONE', #48140, 0.1000000000000000472 ) ;
#37680=DIRECTION ( 'NONE',  ( -4.274815082592931898E-19, -0.9999939076577903929, -0.003490651415223739937 ) ) ;
#37681=DIRECTION ( 'NONE',  ( 0.000000000000000000, -0.000000000000000000, 1.000000000000000000 ) ) ;
#37682=CARTESIAN_POINT ( 'NONE',  ( -8.350000000000012079, 12.50000000000000000, -1.472243186433550122 ) ) ;
#37683=CARTESIAN_POINT ( 'NONE',  ( -8.350000000000008527, 2.500000000000000000, 5.902370205355745192 ) ) ;
#37684=AXIS2_PLACEMENT_3D ( 'NONE', #93184, #44066, #92517 ) ;
#37685=CIRCLE ( 'NONE', #127565, 0.09999999999999982514 ) ;
#37686=EDGE_LOOP ( 'NONE', ( #40307, #53339, #125025, #90609 ) ) ;
#37687=ORIENTED_EDGE ( 'NONE', *, *, #24616, .F. ) ;
#37689=ORIENTED_EDGE ( 'NONE', *, *, #42302, .F. ) ;
#37690=EDGE_LOOP ( 'NONE', ( #91030, #20740 ) ) ;
#37691=DIRECTION ( 'NONE',  ( 0.000000000000000000, 0.000000000000000000, 1.000000000000000000 ) ) ;
#37692=CARTESIAN_POINT ( 'NONE',  ( 0.8499999999999553468, 2.500000000000000000, 1.372243186433545370 ) ) ;
#37693=ORIENTED_EDGE ( 'NONE', *, *, #74186, .F. ) ;
#37694=FACE_BOUND ( 'NONE', #37498, .T. ) ;
#37695=CARTESIAN_POINT ( 'NONE',  ( 4.149999999999936406, 12.50000000000000000, 6.495190528383297135 ) ) ;
#37696=CIRCLE ( 'NONE', #25074, 0.06509327318403745899 ) ;
#37697=FACE_OUTER_BOUND ( 'NONE', #60050, .T. ) ;
#37699=FACE_OUTER_BOUND ( 'NONE', #80819, .T. ) ;
#37700=CARTESIAN_POINT ( 'NONE',  ( 11.24999999999994493, 12.50000000000000000, -2.165063509461101710 ) ) ;
#37701=ORIENTED_EDGE ( 'NONE', *, *, #75144, .T. ) ;
#37702=CARTESIAN_POINT ( 'NONE',  ( -1.650000000000034328, 12.50000000000000000, -2.857883832488653741 ) ) ;
#37703=EDGE_LOOP ( 'NONE', ( #43721, #45319 ) ) ;
#37704=EDGE_LOOP ( 'NONE', ( #75417, #15193, #118937, #51004 ) ) ;
#37706=DIRECTION ( 'NONE',  ( 0.000000000000000000, 0.000000000000000000, -1.000000000000000000 ) ) ;
#37707=CARTESIAN_POINT ( 'NONE',  ( 13.74999999999993072, 12.50000000000000000, -2.165063509461101710 ) ) ;
#37708=DIRECTION ( 'NONE',  ( -0.000000000000000000, -1.000000000000000000, -0.000000000000000000 ) ) ;
#37709=ORIENTED_EDGE ( 'NONE', *, *, #22655, .F. ) ;
#37710=DIRECTION ( 'NONE',  ( -0.000000000000000000, 1.000000000000000000, -0.000000000000000000 ) ) ;
#37711=VECTOR ( 'NONE', #115806, 1000.000000000000000 ) ;
#37712=EDGE_CURVE ( 'NONE', #116743, #118512, #95340, .T. ) ;
#37713=CARTESIAN_POINT ( 'NONE',  ( 14.34999999999989306, 2.500000000000000000, -2.411473670974877859 ) ) ;
#37714=CONICAL_SURFACE ( 'NONE', #41926, 0.1000000000000002554, 0.003490658503988666988 ) ;
#37715=DIRECTION ( 'NONE',  ( 0.000000000000000000, 0.000000000000000000, 1.000000000000000000 ) ) ;
#37717=CARTESIAN_POINT ( 'NONE',  ( -1.850000000000033840, 2.500000000000000000, 6.741600689897071952 ) ) ;
#37718=CARTESIAN_POINT ( 'NONE',  ( 2.099999999999948574, 2.500000000000000000, 3.537306695894645081 ) ) ;
#37719=EDGE_CURVE ( 'NONE', #7038, #13274, #11268, .T. ) ;
#37720=CARTESIAN_POINT ( 'NONE',  ( -4.400000000000025224, 12.50000000000000000, 0.4115034346978109769 ) ) ;
#37721=EDGE_CURVE ( 'NONE', #64904, #116433, #82608, .T. ) ;
#37722=ORIENTED_EDGE ( 'NONE', *, *, #32378, .F. ) ;
#37723=LINE ( 'NONE', #67143, #100631 ) ;
#37724=EDGE_LOOP ( 'NONE', ( #2338, #93113, #66190, #51102 ) ) ;
#37725=EDGE_LOOP ( 'NONE', ( #64706, #42635, #115522, #126990 ) ) ;
#37726=CARTESIAN_POINT ( 'NONE',  ( -12.69999999999999396, 12.50000000000000000, -3.983716857408423628 ) ) ;
#37727=EDGE_CURVE ( 'NONE', #127628, #93079, #103529, .T. ) ;
#37728=EDGE_CURVE ( 'NONE', #89461, #129332, #47232, .T. ) ;
#37729=FACE_OUTER_BOUND ( 'NONE', #74583, .T. ) ;
#37730=DIRECTION ( 'NONE',  ( -0.000000000000000000, -1.000000000000000000, -0.000000000000000000 ) ) ;
#37731=EDGE_CURVE ( 'NONE', #26373, #57597, #113333, .T. ) ;
#37732=EDGE_LOOP ( 'NONE', ( #39375, #78965 ) ) ;
#37733=VERTEX_POINT ( 'NONE', #52479 ) ;
#37734=VECTOR ( 'NONE', #24262, 1000.000000000000000 ) ;
#37735=DIRECTION ( 'NONE',  ( 0.000000000000000000, 0.000000000000000000, 1.000000000000000000 ) ) ;
#37736=CONICAL_SURFACE ( 'NONE', #112949, 0.09999999999999982514, 0.003490658503988666988 ) ;
#37737=CARTESIAN_POINT ( 'NONE',  ( -13.14999999999999147, 2.500000000000000000, -2.511473670974875727 ) ) ;
#37738=DIRECTION ( 'NONE',  ( 0.000000000000000000, 1.000000000000000000, 0.000000000000000000 ) ) ;
#37739=ORIENTED_EDGE ( 'NONE', *, *, #99809, .F. ) ;
#37740=ORIENTED_EDGE ( 'NONE', *, *, #24299, .T. ) ;
#37741=CARTESIAN_POINT ( 'NONE',  ( 10.64999999999991331, 2.500000000000000000, 6.048780366869521252 ) ) ;
#37742=AXIS2_PLACEMENT_3D ( 'NONE', #43793, #61494, #13649 ) ;
#37743=ORIENTED_EDGE ( 'NONE', *, *, #30138, .F. ) ;
#37744=DIRECTION ( 'NONE',  ( 0.000000000000000000, 0.000000000000000000, 1.000000000000000000 ) ) ;
#37745=DIRECTION ( 'NONE',  ( 0.000000000000000000, 0.000000000000000000, 1.000000000000000000 ) ) ;
#37746=ORIENTED_EDGE ( 'NONE', *, *, #38818, .F. ) ;
#37747=CARTESIAN_POINT ( 'NONE',  ( 4.599999999999940137, 2.500000000000000000, -4.230127018922201998 ) ) ;
#37748=DIRECTION ( 'NONE',  ( 0.000000000000000000, -0.9999939076577903929, 0.003490651415223739937 ) ) ;
#37750=CARTESIAN_POINT ( 'NONE',  ( -9.800000000000006040, 12.50000000000000000, 4.676537180435972552 ) ) ;
#37751=CARTESIAN_POINT ( 'NONE',  ( -8.550000000000011369, 2.500000000000000000, -2.611473670974877592 ) ) ;
#37753=DIRECTION ( 'NONE',  ( 0.000000000000000000, 1.000000000000000000, 0.000000000000000000 ) ) ;
#37754=ORIENTED_EDGE ( 'NONE', *, *, #124478, .F. ) ;
#37755=EDGE_LOOP ( 'NONE', ( #61891, #37044, #51594, #112638 ) ) ;
#37756=DIRECTION ( 'NONE',  ( 0.000000000000000000, 0.000000000000000000, -1.000000000000000000 ) ) ;
#37757=DIRECTION ( 'NONE',  ( -4.274815082592931898E-19, -0.9999939076577903929, -0.003490651415223739937 ) ) ;
#37758=DIRECTION ( 'NONE',  ( 0.000000000000000000, -0.000000000000000000, 1.000000000000000000 ) ) ;
#37759=DIRECTION ( 'NONE',  ( -0.000000000000000000, -1.000000000000000000, -0.000000000000000000 ) ) ;
#37760=CARTESIAN_POINT ( 'NONE',  ( -5.600000000000020073, 2.500000000000000000, 4.083716857408421497 ) ) ;
#37761=PLANE ( 'NONE',  #77940 ) ;
#37762=CARTESIAN_POINT ( 'NONE',  ( 16.32360635139512794, 2.500000000000000000, -4.874197684301369016 ) ) ;
#37763=CARTESIAN_POINT ( 'NONE',  ( -8.950000000000009948, 12.50000000000000000, -6.841600689897072485 ) ) ;
#37764=CARTESIAN_POINT ( 'NONE',  ( -4.999999999999986677, 12.50000000000000000, 0.06509327318403515528 ) ) ;
#37765=CONICAL_SURFACE ( 'NONE', #121375, 0.09999999999999982514, 0.003490658503988666988 ) ;
#37766=EDGE_CURVE ( 'NONE', #62255, #54077, #1447, .T. ) ;
#37767=AXIS2_PLACEMENT_3D ( 'NONE', #31020, #82019, #72220 ) ;
#37768=ADVANCED_FACE ( 'NONE', ( #112706 ), #112064, .T. ) ;
#37769=VECTOR ( 'NONE', #2970, 1000.000000000000000 ) ;
#37770=ADVANCED_FACE ( 'NONE', ( #23033 ), #112060, .T. ) ;
#37771=DIRECTION ( 'NONE',  ( 0.000000000000000000, 0.000000000000000000, 1.000000000000000000 ) ) ;
#37772=CIRCLE ( 'NONE', #110911, 0.1000000000000000472 ) ;
#37773=VERTEX_POINT ( 'NONE', #81934 ) ;
#37774=EDGE_CURVE ( 'NONE', #93396, #37336, #101602, .T. ) ;
#37775=DIRECTION ( 'NONE',  ( -0.000000000000000000, -1.000000000000000000, -0.000000000000000000 ) ) ;
#37776=ADVANCED_FACE ( 'NONE', ( #83251 ), #105890, .T. ) ;
#37777=DIRECTION ( 'NONE',  ( 0.000000000000000000, 0.000000000000000000, -1.000000000000000000 ) ) ;
#37778=DIRECTION ( 'NONE',  ( 0.000000000000000000, -0.000000000000000000, 1.000000000000000000 ) ) ;
#37779=DIRECTION ( 'NONE',  ( 0.000000000000000000, 0.000000000000000000, 1.000000000000000000 ) ) ;
#37780=CARTESIAN_POINT ( 'NONE',  ( 1.899999999999949507, 12.50000000000000000, 3.918623584224383727 ) ) ;
#37781=VERTEX_POINT ( 'NONE', #73407 ) ;
#37782=EDGE_CURVE ( 'NONE', #77609, #91178, #59863, .T. ) ;
#37783=CARTESIAN_POINT ( 'NONE',  ( -0.4000000000000392131, 12.50000000000000000, -4.395220292106239768 ) ) ;
#37784=EDGE_CURVE ( 'NONE', #81286, #122177, #93282, .T. ) ;
#37785=DIRECTION ( 'NONE',  ( 0.000000000000000000, -0.000000000000000000, 1.000000000000000000 ) ) ;
#37786=DIRECTION ( 'NONE',  ( 0.000000000000000000, 0.000000000000000000, 1.000000000000000000 ) ) ;
#37787=VERTEX_POINT ( 'NONE', #4019 ) ;
#37788=EDGE_CURVE ( 'NONE', #108866, #39483, #95431, .T. ) ;
#37789=ORIENTED_EDGE ( 'NONE', *, *, #111177, .F. ) ;
#37790=VERTEX_POINT ( 'NONE', #111389 ) ;
#37791=ORIENTED_EDGE ( 'NONE', *, *, #91416, .F. ) ;
#37792=ORIENTED_EDGE ( 'NONE', *, *, #98150, .T. ) ;
#37793=DIRECTION ( 'NONE',  ( -4.274815082592931898E-19, -0.9999939076577903929, -0.003490651415223739937 ) ) ;
#37794=DIRECTION ( 'NONE',  ( 0.000000000000000000, 1.000000000000000000, 0.000000000000000000 ) ) ;
#37795=DIRECTION ( 'NONE',  ( 0.000000000000000000, 1.000000000000000000, 0.000000000000000000 ) ) ;
#37796=CARTESIAN_POINT ( 'NONE',  ( 5.199999999999935341, 2.500000000000000000, -0.2464101615137783419 ) ) ;
#37797=CIRCLE ( 'NONE', #77504, 0.1000000000000002554 ) ;
#37799=CIRCLE ( 'NONE', #121415, 0.06509327318403741736 ) ;
#37800=LINE ( 'NONE', #126829, #96279 ) ;
#37801=ORIENTED_EDGE ( 'NONE', *, *, #115587, .T. ) ;
#37802=DIRECTION ( 'NONE',  ( -0.000000000000000000, 1.000000000000000000, -0.000000000000000000 ) ) ;
#37803=CARTESIAN_POINT ( 'NONE',  ( 14.38463633427091892, -1.499999999999742428, -7.683002070838238495 ) ) ;
#37804=DIRECTION ( 'NONE',  ( 0.000000000000000000, 0.000000000000000000, -1.000000000000000000 ) ) ;
#37805=CARTESIAN_POINT ( 'NONE',  ( 12.89999999999990266, 2.500000000000000000, 3.537306695894645081 ) ) ;
#37806=DIRECTION ( 'NONE',  ( 0.000000000000000000, 0.000000000000000000, 1.000000000000000000 ) ) ;
#37807=AXIS2_PLACEMENT_3D ( 'NONE', #92048, #2355, #42318 ) ;
#37808=ORIENTED_EDGE ( 'NONE', *, *, #88399, .F. ) ;
#37809=AXIS2_PLACEMENT_3D ( 'NONE', #100213, #9896, #99581 ) ;
#37810=EDGE_LOOP ( 'NONE', ( #100343, #74445 ) ) ;
#37811=ORIENTED_EDGE ( 'NONE', *, *, #87661, .T. ) ;
#37812=ORIENTED_EDGE ( 'NONE', *, *, #102449, .F. ) ;
#37813=CARTESIAN_POINT ( 'NONE',  ( 13.14999999999990088, 2.500000000000000000, 1.818653347947321475 ) ) ;
#37814=LINE ( 'NONE', #18808, #51950 ) ;
#37815=CARTESIAN_POINT ( 'NONE',  ( -4.119968255444916849E-14, 2.500000000000000000, 3.637306695894644726 ) ) ;
#37816=FACE_BOUND ( 'NONE', #68132, .T. ) ;
#37817=CARTESIAN_POINT ( 'NONE',  ( 0.6499999999999561684, 2.500000000000000000, -2.411473670974877859 ) ) ;
#37818=CARTESIAN_POINT ( 'NONE',  ( -3.350000000000032507, 2.500000000000000000, -6.495190528383302464 ) ) ;
#37819=CARTESIAN_POINT ( 'NONE',  ( -2.100000000000034284, 2.500000000000000000, -2.385244779468109755E-15 ) ) ;
#37820=CARTESIAN_POINT ( 'NONE',  ( 6.449999999999928235, 2.500000000000000000, 2.411473670974873862 ) ) ;
#37821=AXIS2_PLACEMENT_3D ( 'NONE', #39905, #90251, #30087 ) ;
#37822=CONICAL_SURFACE ( 'NONE', #90034, 0.1000000000000002554, 0.003490658503988666988 ) ;
#37823=EDGE_CURVE ( 'NONE', #88819, #124287, #55708, .T. ) ;
#37825=CARTESIAN_POINT ( 'NONE',  ( 9.599999999999914380, 2.500000000000000000, -5.122947341949753763 ) ) ;
#37826=DIRECTION ( 'NONE',  ( 0.000000000000000000, 0.000000000000000000, 1.000000000000000000 ) ) ;
#37827=CONICAL_SURFACE ( 'NONE', #71267, 0.09999999999999982514, 0.003490658503988666988 ) ;
#37828=CARTESIAN_POINT ( 'NONE',  ( 3.149999999999946176, 2.500000000000000000, -6.841600689897077814 ) ) ;
#37829=ORIENTED_EDGE ( 'NONE', *, *, #24437, .T. ) ;
#37830=CIRCLE ( 'NONE', #100520, 0.1000000000000002554 ) ;
#37831=ORIENTED_EDGE ( 'NONE', *, *, #47397, .T. ) ;
#37833=EDGE_LOOP ( 'NONE', ( #113713, #112076, #44669, #41596 ) ) ;
#37834=DIRECTION ( 'NONE',  ( 0.000000000000000000, -0.000000000000000000, 1.000000000000000000 ) ) ;
#37835=FACE_BOUND ( 'NONE', #3401, .T. ) ;
#37836=LINE ( 'NONE', #128833, #122998 ) ;
#37837=ORIENTED_EDGE ( 'NONE', *, *, #30085, .T. ) ;
#37838=CARTESIAN_POINT ( 'NONE',  ( -2.499999999999996003, 2.500000000000000000, -2.276824562219559311E-15 ) ) ;
#37839=LINE ( 'NONE', #77751, #129401 ) ;
#37840=CARTESIAN_POINT ( 'NONE',  ( -14.34999999999998543, 12.50000000000000000, -1.818653347947323695 ) ) ;
#37841=ORIENTED_EDGE ( 'NONE', *, *, #77747, .T. ) ;
#37842=CARTESIAN_POINT ( 'NONE',  ( -2.950000000000029932, 2.500000000000000000, -2.065063509461102065 ) ) ;
#37843=DIRECTION ( 'NONE',  ( -0.000000000000000000, 1.000000000000000000, -0.000000000000000000 ) ) ;
#37844=VERTEX_POINT ( 'NONE', #21749 ) ;
#37845=CIRCLE ( 'NONE', #2327, 0.09999999999999999167 ) ;
#37846=ORIENTED_EDGE ( 'NONE', *, *, #67851, .T. ) ;
#37847=AXIS2_PLACEMENT_3D ( 'NONE', #115318, #34237, #54490 ) ;
#37848=DIRECTION ( 'NONE',  ( -0.000000000000000000, -1.000000000000000000, -0.000000000000000000 ) ) ;
#37849=DIRECTION ( 'NONE',  ( 0.000000000000000000, 0.000000000000000000, 1.000000000000000000 ) ) ;
#37850=EDGE_CURVE ( 'NONE', #98051, #4680, #61682, .T. ) ;
#37851=DIRECTION ( 'NONE',  ( -0.000000000000000000, -1.000000000000000000, -0.000000000000000000 ) ) ;
#37852=AXIS2_PLACEMENT_3D ( 'NONE', #27470, #67374, #47784 ) ;
#37853=FACE_OUTER_BOUND ( 'NONE', #76834, .T. ) ;
#37854=VERTEX_POINT ( 'NONE', #26259 ) ;
#37855=DIRECTION ( 'NONE',  ( -0.000000000000000000, 1.000000000000000000, -0.000000000000000000 ) ) ;
#37856=VERTEX_POINT ( 'NONE', #56343 ) ;
#37857=AXIS2_PLACEMENT_3D ( 'NONE', #129356, #97928, #128719 ) ;
#37858=ORIENTED_EDGE ( 'NONE', *, *, #80176, .T. ) ;
#37859=ADVANCED_FACE ( 'NONE', ( #18839 ), #39030, .T. ) ;
#37860=DIRECTION ( 'NONE',  ( 0.000000000000000000, 0.000000000000000000, -1.000000000000000000 ) ) ;
#37861=ADVANCED_FACE ( 'NONE', ( #113992 ), #114212, .T. ) ;
#37862=ORIENTED_EDGE ( 'NONE', *, *, #29029, .F. ) ;
#37863=DIRECTION ( 'NONE',  ( 0.000000000000000000, 0.000000000000000000, 1.000000000000000000 ) ) ;
#37864=FACE_BOUND ( 'NONE', #129466, .T. ) ;
#37865=ORIENTED_EDGE ( 'NONE', *, *, #19775, .F. ) ;
#37866=DIRECTION ( 'NONE',  ( 0.000000000000000000, -0.9999939076577903929, 0.003490651415223739937 ) ) ;
#37867=VERTEX_POINT ( 'NONE', #74062 ) ;
#37868=DIRECTION ( 'NONE',  ( 0.000000000000000000, -1.000000000000000000, 0.000000000000000000 ) ) ;
#37869=CARTESIAN_POINT ( 'NONE',  ( -11.64999999999999680, 2.500000000000000000, -2.265063509461097802 ) ) ;
#37870=EDGE_CURVE ( 'NONE', #120381, #98606, #58778, .T. ) ;
#37871=ADVANCED_FACE ( 'NONE', ( #75990 ), #5527, .T. ) ;
#37872=CARTESIAN_POINT ( 'NONE',  ( -9.200000000000006395, 12.50000000000000000, -2.385244779468109755E-15 ) ) ;
#37873=EDGE_CURVE ( 'NONE', #2890, #74712, #128907, .T. ) ;
#37874=DIRECTION ( 'NONE',  ( 0.000000000000000000, 0.000000000000000000, 1.000000000000000000 ) ) ;
#37875=EDGE_CURVE ( 'NONE', #84780, #86820, #48971, .T. ) ;
#37876=EDGE_CURVE ( 'NONE', #27877, #54474, #64869, .T. ) ;
#37877=DIRECTION ( 'NONE',  ( 0.000000000000000000, 0.000000000000000000, 1.000000000000000000 ) ) ;
#37878=EDGE_LOOP ( 'NONE', ( #9663, #86161 ) ) ;
#37879=VERTEX_POINT ( 'NONE', #54412 ) ;
#37880=AXIS2_PLACEMENT_3D ( 'NONE', #78467, #67966, #128195 ) ;
#37881=DIRECTION ( 'NONE',  ( -0.000000000000000000, -1.000000000000000000, -0.000000000000000000 ) ) ;
#37882=CARTESIAN_POINT ( 'NONE',  ( 18.29531403502771525, -0.5011766475904755325, 4.780851392375801368 ) ) ;
#37883=CARTESIAN_POINT ( 'NONE',  ( -5.200000000000025935, 2.500000000000000000, -3.883716857408426648 ) ) ;
#37884=ORIENTED_EDGE ( 'NONE', *, *, #124967, .T. ) ;
#37885=ORIENTED_EDGE ( 'NONE', *, *, #66007, .T. ) ;
#37886=ORIENTED_EDGE ( 'NONE', *, *, #74556, .F. ) ;
#37887=EDGE_CURVE ( 'NONE', #27095, #86001, #97484, .T. ) ;
#37888=CARTESIAN_POINT ( 'NONE',  ( 12.09999999999990550, 2.500000000000000000, 5.022947341949748790 ) ) ;
#37889=LINE ( 'NONE', #80408, #4657 ) ;
#37890=CONICAL_SURFACE ( 'NONE', #2354, 0.1000000000000002554, 0.003490658503988666988 ) ;
#37891=DIRECTION ( 'NONE',  ( -0.000000000000000000, 1.000000000000000000, -0.000000000000000000 ) ) ;
#37892=CARTESIAN_POINT ( 'NONE',  ( -0.4500000000000397571, 2.500000000000000000, -6.495190528383302464 ) ) ;
#37894=DIRECTION ( 'NONE',  ( 0.000000000000000000, 0.000000000000000000, -1.000000000000000000 ) ) ;
#37895=DIRECTION ( 'NONE',  ( 0.000000000000000000, 0.000000000000000000, -1.000000000000000000 ) ) ;
#37896=DIRECTION ( 'NONE',  ( -0.000000000000000000, 1.000000000000000000, -0.000000000000000000 ) ) ;
#37897=AXIS2_PLACEMENT_3D ( 'NONE', #101010, #121299, #61755 ) ;
#37898=VERTEX_POINT ( 'NONE', #5307 ) ;
#37899=CIRCLE ( 'NONE', #125703, 0.09999999999999982514 ) ;
#37901=DIRECTION ( 'NONE',  ( 0.000000000000000000, 0.000000000000000000, 1.000000000000000000 ) ) ;
#37902=CARTESIAN_POINT ( 'NONE',  ( -1.450000000000035483, 2.500000000000000000, 1.918653347947321564 ) ) ;
#37903=VERTEX_POINT ( 'NONE', #95000 ) ;
#37904=VERTEX_POINT ( 'NONE', #94329 ) ;
#37906=CARTESIAN_POINT ( 'NONE',  ( 7.499999999999961808, 2.500000000000000000, 4.330127018922196314 ) ) ;
#37907=FACE_OUTER_BOUND ( 'NONE', #25040, .T. ) ;
#37908=CONICAL_SURFACE ( 'NONE', #25368, 0.09999999999999999167, 0.003490658503988666988 ) ;
#37910=VECTOR ( 'NONE', #93999, 1000.000000000000000 ) ;
#37911=CARTESIAN_POINT ( 'NONE',  ( 3.149999999999942624, 2.500000000000000000, 6.048780366869521252 ) ) ;
#37912=DIRECTION ( 'NONE',  ( -0.000000000000000000, 1.000000000000000000, -0.000000000000000000 ) ) ;
#37913=CARTESIAN_POINT ( 'NONE',  ( -11.64999999999999680, 2.500000000000000000, 2.957883832488649389 ) ) ;
#37914=AXIS2_PLACEMENT_3D ( 'NONE', #93331, #63220, #20725 ) ;
#37915=ORIENTED_EDGE ( 'NONE', *, *, #18699, .F. ) ;
#37916=DIRECTION ( 'NONE',  ( 0.000000000000000000, 1.000000000000000000, 0.000000000000000000 ) ) ;
#37917=EDGE_CURVE ( 'NONE', #117010, #54102, #104167, .T. ) ;
#37918=EDGE_CURVE ( 'NONE', #71367, #100917, #128167, .T. ) ;
#37919=CONICAL_SURFACE ( 'NONE', #113126, 0.09999999999999999167, 0.003490658503988666988 ) ;
#37920=ADVANCED_FACE ( 'NONE', ( #65522 ), #66170, .T. ) ;
#37921=DIRECTION ( 'NONE',  ( -0.000000000000000000, -1.000000000000000000, -0.000000000000000000 ) ) ;
#37922=ORIENTED_EDGE ( 'NONE', *, *, #28176, .F. ) ;
#37923=EDGE_CURVE ( 'NONE', #84687, #36770, #82918, .T. ) ;
#37924=AXIS2_PLACEMENT_3D ( 'NONE', #70204, #40103, #108178 ) ;
#37925=CIRCLE ( 'NONE', #111054, 0.06509327318403745899 ) ;
#37926=ORIENTED_EDGE ( 'NONE', *, *, #99591, .T. ) ;
#37927=VERTEX_POINT ( 'NONE', #44604 ) ;
#37928=EDGE_CURVE ( 'NONE', #89300, #73117, #11800, .T. ) ;
#37929=VERTEX_POINT ( 'NONE', #105462 ) ;
#37930=CARTESIAN_POINT ( 'NONE',  ( -8.100000000000013856, 2.500000000000000000, 0.2464101615137736789 ) ) ;
#37931=FACE_OUTER_BOUND ( 'NONE', #126179, .T. ) ;
#37932=ADVANCED_FACE ( 'NONE', ( #34803 ), #110017, .T. ) ;
#37933=ORIENTED_EDGE ( 'NONE', *, *, #13087, .T. ) ;
#37934=EDGE_CURVE ( 'NONE', #83506, #105517, #76559, .T. ) ;
#37935=CARTESIAN_POINT ( 'NONE',  ( 4.549999999999939426, 2.500000000000000000, -2.165063509461101710 ) ) ;
#37936=LINE ( 'NONE', #46454, #54928 ) ;
#37937=EDGE_CURVE ( 'NONE', #885, #125076, #45259, .T. ) ;
#37938=DIRECTION ( 'NONE',  ( 0.000000000000000000, 0.000000000000000000, -1.000000000000000000 ) ) ;
#37939=DIRECTION ( 'NONE',  ( 0.000000000000000000, 0.000000000000000000, 1.000000000000000000 ) ) ;
#37940=ORIENTED_EDGE ( 'NONE', *, *, #92396, .T. ) ;
#37941=CARTESIAN_POINT ( 'NONE',  ( 8.149999999999920419, 12.50000000000000000, 6.841600689897072485 ) ) ;
#37943=CARTESIAN_POINT ( 'NONE',  ( 8.949999999999921130, 2.500000000000000000, 1.818653347947321475 ) ) ;
#37944=VERTEX_POINT ( 'NONE', #101278 ) ;
#37945=ORIENTED_EDGE ( 'NONE', *, *, #1919, .F. ) ;
#37946=ORIENTED_EDGE ( 'NONE', *, *, #7591, .T. ) ;
#37947=AXIS2_PLACEMENT_3D ( 'NONE', #11076, #619, #40586 ) ;
#37948=CARTESIAN_POINT ( 'NONE',  ( 13.09999999999990195, 2.500000000000000000, 4.576537180435972019 ) ) ;
#37949=AXIS2_PLACEMENT_3D ( 'NONE', #31485, #103933, #71384 ) ;
#37950=CIRCLE ( 'NONE', #111078, 0.06509327318403745899 ) ;
#37951=CARTESIAN_POINT ( 'NONE',  ( -2.100000000000033840, 2.500000000000000000, 5.022947341949748790 ) ) ;
#37952=CIRCLE ( 'NONE', #67166, 0.1000000000000000472 ) ;
#37953=AXIS2_PLACEMENT_3D ( 'NONE', #111452, #112765, #10658 ) ;
#37954=EDGE_LOOP ( 'NONE', ( #90743, #62058, #71111, #17246 ) ) ;
#37955=CARTESIAN_POINT ( 'NONE',  ( -3.150000000000030109, 2.500000000000000000, 1.818653347947321475 ) ) ;
#37956=DIRECTION ( 'NONE',  ( 0.000000000000000000, 1.000000000000000000, 0.000000000000000000 ) ) ;
#37957=CARTESIAN_POINT ( 'NONE',  ( 3.349999999999945466, 2.500000000000000000, -6.495190528383302464 ) ) ;
#37958=DIRECTION ( 'NONE',  ( 0.000000000000000000, 0.000000000000000000, -1.000000000000000000 ) ) ;
#37959=EDGE_CURVE ( 'NONE', #90001, #128895, #79073, .T. ) ;
#37960=ORIENTED_EDGE ( 'NONE', *, *, #97864, .F. ) ;
#37961=DIRECTION ( 'NONE',  ( 0.000000000000000000, -0.000000000000000000, 1.000000000000000000 ) ) ;
#37962=ORIENTED_EDGE ( 'NONE', *, *, #10352, .F. ) ;
#37963=ORIENTED_EDGE ( 'NONE', *, *, #89935, .T. ) ;
#37964=CARTESIAN_POINT ( 'NONE',  ( -0.6500000000000389910, 12.50000000000000000, -6.148780366869526226 ) ) ;
#37965=PLANE ( 'NONE',  #127618 ) ;
#37966=FACE_BOUND ( 'NONE', #76791, .T. ) ;
#37967=CARTESIAN_POINT ( 'NONE',  ( 17.50000000000000000, 2.500000000000000444, 4.040567763474975926 ) ) ;
#37968=CARTESIAN_POINT ( 'NONE',  ( 8.749999999999953815, 12.50000000000000000, 6.560283801567334372 ) ) ;
#37970=EDGE_CURVE ( 'NONE', #85122, #83523, #116254, .T. ) ;
#37971=ORIENTED_EDGE ( 'NONE', *, *, #52578, .T. ) ;
#37973=CARTESIAN_POINT ( 'NONE',  ( -1.650000000000035660, 12.50000000000000000, 2.857883832488649301 ) ) ;
#37974=LINE ( 'NONE', #64849, #42490 ) ;
#37975=DIRECTION ( 'NONE',  ( 0.000000000000000000, 0.000000000000000000, -1.000000000000000000 ) ) ;
#37976=ORIENTED_EDGE ( 'NONE', *, *, #107530, .T. ) ;
#37977=CIRCLE ( 'NONE', #25433, 0.06509327318403745899 ) ;
#37978=CARTESIAN_POINT ( 'NONE',  ( -6.249999999999984901, 12.50000000000000000, -2.165063509461101710 ) ) ;
#37979=CIRCLE ( 'NONE', #58826, 0.1000000000000002554 ) ;
#37980=CARTESIAN_POINT ( 'NONE',  ( 0.4499999999999569344, 2.500000000000000000, 2.165063509461097713 ) ) ;
#37981=EDGE_LOOP ( 'NONE', ( #4631, #73160, #73517, #60723 ) ) ;
#37982=EDGE_LOOP ( 'NONE', ( #85227, #51048 ) ) ;
#37983=DIRECTION ( 'NONE',  ( -0.000000000000000000, -1.000000000000000000, -0.000000000000000000 ) ) ;
#37984=EDGE_CURVE ( 'NONE', #25471, #41232, #13844, .T. ) ;
#37985=DIRECTION ( 'NONE',  ( 0.000000000000000000, -0.000000000000000000, 1.000000000000000000 ) ) ;
#37986=FACE_BOUND ( 'NONE', #52497, .T. ) ;
#37987=AXIS2_PLACEMENT_3D ( 'NONE', #31377, #33318, #101402 ) ;
#37988=DIRECTION ( 'NONE',  ( 0.000000000000000000, 0.000000000000000000, -1.000000000000000000 ) ) ;
#37989=ORIENTED_EDGE ( 'NONE', *, *, #35738, .T. ) ;
#37990=AXIS2_PLACEMENT_3D ( 'NONE', #66575, #127449, #107142 ) ;
#37991=CARTESIAN_POINT ( 'NONE',  ( -12.69999999999999041, 2.500000000000000000, 3.983716857408420964 ) ) ;
#37992=ORIENTED_EDGE ( 'NONE', *, *, #18333, .T. ) ;
#37993=VERTEX_POINT ( 'NONE', #62009 ) ;
#37994=CARTESIAN_POINT ( 'NONE',  ( -10.60000000000000142, 12.50000000000000000, 3.983716857408420964 ) ) ;
#37997=EDGE_LOOP ( 'NONE', ( #117013, #77267 ) ) ;
#37998=AXIS2_PLACEMENT_3D ( 'NONE', #61311, #103157, #41686 ) ;
#37999=LINE ( 'NONE', #77280, #124190 ) ;
#38000=LINE ( 'NONE', #17702, #97132 ) ;
#38002=CONICAL_SURFACE ( 'NONE', #92367, 0.09999999999999999167, 0.003490658503988666988 ) ;
#38003=CIRCLE ( 'NONE', #40169, 0.06509327318403741736 ) ;
#38004=CONICAL_SURFACE ( 'NONE', #52676, 0.09999999999999982514, 0.003490658503988666988 ) ;
#38005=DIRECTION ( 'NONE',  ( -0.000000000000000000, -1.000000000000000000, -0.000000000000000000 ) ) ;
#38006=CARTESIAN_POINT ( 'NONE',  ( 7.099999999999926814, 2.500000000000000000, -2.276824562219559311E-15 ) ) ;
#38007=AXIS2_PLACEMENT_3D ( 'NONE', #69694, #109629, #8187 ) ;
#38008=ORIENTED_EDGE ( 'NONE', *, *, #103331, .T. ) ;
#38009=EDGE_CURVE ( 'NONE', #17110, #106540, #70302, .T. ) ;
#38011=AXIS2_PLACEMENT_3D ( 'NONE', #43971, #4647, #44607 ) ;
#38012=DIRECTION ( 'NONE',  ( 0.000000000000000000, 0.000000000000000000, 1.000000000000000000 ) ) ;
#38013=DIRECTION ( 'NONE',  ( 0.000000000000000000, 1.000000000000000000, 0.000000000000000000 ) ) ;
#38014=DIRECTION ( 'NONE',  ( -0.000000000000000000, 1.000000000000000000, -0.000000000000000000 ) ) ;
#38015=ORIENTED_EDGE ( 'NONE', *, *, #1235, .T. ) ;
#38016=DIRECTION ( 'NONE',  ( -4.274815082592931898E-19, -0.9999939076577903929, -0.003490651415223739937 ) ) ;
#38017=VERTEX_POINT ( 'NONE', #475 ) ;
#38018=CARTESIAN_POINT ( 'NONE',  ( 1.699999999999951994, 12.50000000000000000, -4.265033745738164406 ) ) ;
#38019=ORIENTED_EDGE ( 'NONE', *, *, #69500, .T. ) ;
#38020=DIRECTION ( 'NONE',  ( -0.000000000000000000, 1.000000000000000000, -0.000000000000000000 ) ) ;
#38021=DIRECTION ( 'NONE',  ( 0.000000000000000000, 1.000000000000000000, 0.000000000000000000 ) ) ;
#38023=DIRECTION ( 'NONE',  ( 0.000000000000000000, 0.000000000000000000, 1.000000000000000000 ) ) ;
#38024=VERTEX_POINT ( 'NONE', #10930 ) ;
#38026=DIRECTION ( 'NONE',  ( -0.000000000000000000, 1.000000000000000000, -0.000000000000000000 ) ) ;
#38027=EDGE_CURVE ( 'NONE', #105557, #76276, #120471, .T. ) ;
#38028=EDGE_CURVE ( 'NONE', #69282, #116043, #90810, .T. ) ;
#38030=CARTESIAN_POINT ( 'NONE',  ( 10.79999999999991012, 12.50000000000000000, -4.330127018922201643 ) ) ;
#38031=EDGE_CURVE ( 'NONE', #84244, #74651, #18052, .T. ) ;
#38032=EDGE_CURVE ( 'NONE', #12562, #25677, #80994, .T. ) ;
#38033=CARTESIAN_POINT ( 'NONE',  ( 7.499999999999961808, 12.50000000000000000, -4.395220292106239768 ) ) ;
#38034=ORIENTED_EDGE ( 'NONE', *, *, #15974, .T. ) ;
#38035=ORIENTED_EDGE ( 'NONE', *, *, #104116, .F. ) ;
#38036=CARTESIAN_POINT ( 'NONE',  ( -14.19999999999998685, 12.50000000000000000, 0.06509327318403732021 ) ) ;
#38037=EDGE_CURVE ( 'NONE', #13161, #75848, #118980, .T. ) ;
#38038=ORIENTED_EDGE ( 'NONE', *, *, #79452, .T. ) ;
#38039=DIRECTION ( 'NONE',  ( 0.000000000000000000, 0.000000000000000000, -1.000000000000000000 ) ) ;
#38040=VECTOR ( 'NONE', #19399, 1000.000000000000000 ) ;
#38041=AXIS2_PLACEMENT_3D ( 'NONE', #110667, #12464, #52398 ) ;
#38042=ORIENTED_EDGE ( 'NONE', *, *, #98032, .F. ) ;
#38043=VERTEX_POINT ( 'NONE', #29322 ) ;
#38044=EDGE_LOOP ( 'NONE', ( #61915, #73781 ) ) ;
#38045=ADVANCED_FACE ( 'NONE', ( #52178 ), #91451, .T. ) ;
#38046=DIRECTION ( 'NONE',  ( 0.000000000000000000, 1.000000000000000000, 0.000000000000000000 ) ) ;
#38047=EDGE_CURVE ( 'NONE', #36161, #32820, #80775, .T. ) ;
#38048=DIRECTION ( 'NONE',  ( 0.000000000000000000, -0.9999939076577903929, 0.003490651415223739937 ) ) ;
#38049=EDGE_CURVE ( 'NONE', #79899, #63390, #124682, .T. ) ;
#38050=CIRCLE ( 'NONE', #59285, 0.06509327318403745899 ) ;
#38051=CARTESIAN_POINT ( 'NONE',  ( -11.69999999999999929, 2.500000000000000000, -4.330127018922198978 ) ) ;
#38052=AXIS2_PLACEMENT_3D ( 'NONE', #118851, #79581, #119488 ) ;
#38054=DIRECTION ( 'NONE',  ( 0.000000000000000000, 0.000000000000000000, 1.000000000000000000 ) ) ;
#38055=DIRECTION ( 'NONE',  ( -0.000000000000000000, -1.000000000000000000, -0.000000000000000000 ) ) ;
#38056=DIRECTION ( 'NONE',  ( 0.000000000000000000, 0.000000000000000000, 1.000000000000000000 ) ) ;
#38057=LINE ( 'NONE', #23896, #80277 ) ;
#38058=CIRCLE ( 'NONE', #33841, 0.06509327318403745899 ) ;
#38060=EDGE_CURVE ( 'NONE', #77627, #78283, #78816, .T. ) ;
#38061=DIRECTION ( 'NONE',  ( 0.000000000000000000, -0.000000000000000000, 1.000000000000000000 ) ) ;
#38062=VECTOR ( 'NONE', #68422, 1000.000000000000000 ) ;
#38063=ORIENTED_EDGE ( 'NONE', *, *, #81010, .F. ) ;
#38064=VERTEX_POINT ( 'NONE', #111068 ) ;
#38065=EDGE_LOOP ( 'NONE', ( #26331, #125753, #62093, #13226 ) ) ;
#38066=ORIENTED_EDGE ( 'NONE', *, *, #112345, .T. ) ;
#38067=CARTESIAN_POINT ( 'NONE',  ( -14.54999999999998472, 12.50000000000000000, 2.099970236277064028 ) ) ;
#38068=ORIENTED_EDGE ( 'NONE', *, *, #50019, .T. ) ;
#38069=ORIENTED_EDGE ( 'NONE', *, *, #125101, .F. ) ;
#38070=CARTESIAN_POINT ( 'NONE',  ( 0.6499999999999561684, 12.50000000000000000, 1.818653347947321475 ) ) ;
#38071=DIRECTION ( 'NONE',  ( 0.000000000000000000, -0.9999939076577903929, 0.003490651415223739937 ) ) ;
#38072=DIRECTION ( 'NONE',  ( -0.000000000000000000, 1.000000000000000000, -0.000000000000000000 ) ) ;
#38073=CARTESIAN_POINT ( 'NONE',  ( 8.349999999999923261, 12.50000000000000000, -5.802370205355749988 ) ) ;
#38074=DIRECTION ( 'NONE',  ( 0.000000000000000000, 0.000000000000000000, 1.000000000000000000 ) ) ;
#38075=EDGE_LOOP ( 'NONE', ( #78266, #21363 ) ) ;
#38076=FACE_OUTER_BOUND ( 'NONE', #12054, .T. ) ;
#38077=CIRCLE ( 'NONE', #44325, 0.1000000000000002554 ) ;
#38078=CIRCLE ( 'NONE', #111117, 0.1000000000000002554 ) ;
#38079=ORIENTED_EDGE ( 'NONE', *, *, #115587, .F. ) ;
#38080=LINE ( 'NONE', #8590, #113616 ) ;
#38081=ORIENTED_EDGE ( 'NONE', *, *, #14691, .F. ) ;
#38082=DIRECTION ( 'NONE',  ( 0.000000000000000000, -0.9999939076577903929, 0.003490651415223739937 ) ) ;
#38083=ORIENTED_EDGE ( 'NONE', *, *, #106164, .F. ) ;
#38084=ORIENTED_EDGE ( 'NONE', *, *, #58628, .F. ) ;
#38085=AXIS2_PLACEMENT_3D ( 'NONE', #112510, #73226, #113140 ) ;
#38086=DIRECTION ( 'NONE',  ( 0.000000000000000000, -0.000000000000000000, 1.000000000000000000 ) ) ;
#38087=DIRECTION ( 'NONE',  ( 0.000000000000000000, 0.000000000000000000, 1.000000000000000000 ) ) ;
#38088=AXIS2_PLACEMENT_3D ( 'NONE', #91337, #92629, #101166 ) ;
#38089=EDGE_CURVE ( 'NONE', #71724, #86890, #76741, .T. ) ;
#38090=CIRCLE ( 'NONE', #104961, 0.1000000000000002554 ) ;
#38092=VECTOR ( 'NONE', #58555, 1000.000000000000000 ) ;
#38093=DIRECTION ( 'NONE',  ( 0.000000000000000000, 0.000000000000000000, 1.000000000000000000 ) ) ;
#38094=ADVANCED_FACE ( 'NONE', ( #21421 ), #59445, .T. ) ;
#38095=DIRECTION ( 'NONE',  ( -4.274815082592931898E-19, -0.9999939076577903929, -0.003490651415223739937 ) ) ;
#38096=EDGE_LOOP ( 'NONE', ( #116159, #101109, #60740, #122606 ) ) ;
#38097=DIRECTION ( 'NONE',  ( 0.000000000000000000, 1.000000000000000000, 0.000000000000000000 ) ) ;
#38098=DIRECTION ( 'NONE',  ( -0.000000000000000000, 1.000000000000000000, -0.000000000000000000 ) ) ;
#38099=DIRECTION ( 'NONE',  ( -0.000000000000000000, 1.000000000000000000, -0.000000000000000000 ) ) ;
#38100=DIRECTION ( 'NONE',  ( 0.000000000000000000, 1.000000000000000000, 0.000000000000000000 ) ) ;
#38101=CONICAL_SURFACE ( 'NONE', #117476, 0.09999999999999982514, 0.003490658503988666988 ) ;
#38102=ADVANCED_FACE ( 'NONE', ( #39799 ), #89260, .T. ) ;
#38103=CIRCLE ( 'NONE', #90305, 0.06509327318403745899 ) ;
#38104=FACE_OUTER_BOUND ( 'NONE', #35623, .T. ) ;
#38105=EDGE_LOOP ( 'NONE', ( #5493, #122382 ) ) ;
#38106=AXIS2_PLACEMENT_3D ( 'NONE', #74215, #62478, #52631 ) ;
#38107=AXIS2_PLACEMENT_3D ( 'NONE', #74739, #114023, #76674 ) ;
#38108=VERTEX_POINT ( 'NONE', #60082 ) ;
#38109=DIRECTION ( 'NONE',  ( 0.000000000000000000, 0.000000000000000000, 1.000000000000000000 ) ) ;
#38110=VECTOR ( 'NONE', #28827, 1000.000000000000000 ) ;
#38111=VERTEX_POINT ( 'NONE', #50251 ) ;
#38112=CARTESIAN_POINT ( 'NONE',  ( -3.350000000000032507, 2.500000000000000000, -6.595190528383302109 ) ) ;
#38113=DIRECTION ( 'NONE',  ( 0.000000000000000000, 1.000000000000000000, 0.000000000000000000 ) ) ;
#38114=VECTOR ( 'NONE', #21590, 1000.000000000000000 ) ;
#38115=EDGE_LOOP ( 'NONE', ( #66383, #44480, #99478, #104848 ) ) ;
#38117=DIRECTION ( 'NONE',  ( 0.000000000000000000, 0.000000000000000000, 1.000000000000000000 ) ) ;
#38118=CARTESIAN_POINT ( 'NONE',  ( 1.849999999999949019, 12.50000000000000000, 6.841600689897072485 ) ) ;
#38119=DIRECTION ( 'NONE',  ( -0.000000000000000000, 1.000000000000000000, -0.000000000000000000 ) ) ;
#38120=ORIENTED_EDGE ( 'NONE', *, *, #102449, .T. ) ;
#38121=CARTESIAN_POINT ( 'NONE',  ( -1.250000000000037526, 2.500000000000000000, -5.702370205355749455 ) ) ;
#38122=DIRECTION ( 'NONE',  ( 0.000000000000000000, -0.000000000000000000, 1.000000000000000000 ) ) ;
#38123=ORIENTED_EDGE ( 'NONE', *, *, #9953, .F. ) ;
#38124=CARTESIAN_POINT ( 'NONE',  ( 1.649999999999951505, 12.50000000000000000, 1.472243186433545459 ) ) ;
#38125=FACE_OUTER_BOUND ( 'NONE', #93564, .T. ) ;
#38126=DIRECTION ( 'NONE',  ( -0.000000000000000000, -1.000000000000000000, -0.000000000000000000 ) ) ;
#38127=ORIENTED_EDGE ( 'NONE', *, *, #123340, .T. ) ;
#38128=CARTESIAN_POINT ( 'NONE',  ( 1.849999999999948130, 2.500000000000000000, 6.048780366869520364 ) ) ;
#38129=CIRCLE ( 'NONE', #81933, 0.1000000000000000472 ) ;
#38130=CIRCLE ( 'NONE', #75673, 0.06509327318403745899 ) ;
#38131=ORIENTED_EDGE ( 'NONE', *, *, #42682, .T. ) ;
#38132=CARTESIAN_POINT ( 'NONE',  ( -12.49999999999995914, 2.500000000000000000, -4.330127018922198978 ) ) ;
#38133=CARTESIAN_POINT ( 'NONE',  ( -4.600000000000024514, 2.500000000000000000, 0.6928203230275494784 ) ) ;
#38134=DIRECTION ( 'NONE',  ( 0.000000000000000000, 1.000000000000000000, 0.000000000000000000 ) ) ;
#38135=VERTEX_POINT ( 'NONE', #55401 ) ;
#38136=AXIS2_PLACEMENT_3D ( 'NONE', #104077, #114522, #65428 ) ;
#38137=LINE ( 'NONE', #117976, #65647 ) ;
#38140=DIRECTION ( 'NONE',  ( 0.000000000000000000, 0.000000000000000000, 1.000000000000000000 ) ) ;
#38141=AXIS2_PLACEMENT_3D ( 'NONE', #100979, #102280, #110794 ) ;
#38142=EDGE_CURVE ( 'NONE', #42165, #32002, #113022, .T. ) ;
#38143=EDGE_LOOP ( 'NONE', ( #119419, #101501 ) ) ;
#38144=LINE ( 'NONE', #19795, #76121 ) ;
#38145=EDGE_CURVE ( 'NONE', #48067, #13926, #41170, .T. ) ;
#38146=VERTEX_POINT ( 'NONE', #105131 ) ;
#38147=CONICAL_SURFACE ( 'NONE', #105032, 0.09999999999999982514, 0.003490658503988666988 ) ;
#38148=DIRECTION ( 'NONE',  ( 0.000000000000000000, 0.000000000000000000, 1.000000000000000000 ) ) ;
#38149=ORIENTED_EDGE ( 'NONE', *, *, #126053, .T. ) ;
#38150=DIRECTION ( 'NONE',  ( -0.000000000000000000, -1.000000000000000000, -0.000000000000000000 ) ) ;
#38151=CARTESIAN_POINT ( 'NONE',  ( 10.39999999999991509, 12.50000000000000000, 0.6928203230275494784 ) ) ;
#38152=ORIENTED_EDGE ( 'NONE', *, *, #53575, .T. ) ;
#38153=EDGE_CURVE ( 'NONE', #5078, #106111, #94031, .T. ) ;
#38154=VERTEX_POINT ( 'NONE', #75041 ) ;
#38155=DIRECTION ( 'NONE',  ( -0.000000000000000000, 1.000000000000000000, -0.000000000000000000 ) ) ;
#38156=DIRECTION ( 'NONE',  ( 0.000000000000000000, 0.000000000000000000, -1.000000000000000000 ) ) ;
#38157=ORIENTED_EDGE ( 'NONE', *, *, #76349, .F. ) ;
#38158=VECTOR ( 'NONE', #18144, 1000.000000000000000 ) ;
#38159=CARTESIAN_POINT ( 'NONE',  ( -4.800000000000022915, 2.500000000000000000, -0.3464101615137783474 ) ) ;
#38161=DIRECTION ( 'NONE',  ( -0.000000000000000000, 1.000000000000000000, -0.000000000000000000 ) ) ;
#38162=CARTESIAN_POINT ( 'NONE',  ( -11.44999999999999929, 12.50000000000000000, -1.818653347947322141 ) ) ;
#38163=DIRECTION ( 'NONE',  ( 0.000000000000000000, 0.000000000000000000, -1.000000000000000000 ) ) ;
#38164=DIRECTION ( 'NONE',  ( -4.274815082592931898E-19, -0.9999939076577903929, -0.003490651415223739937 ) ) ;
#38165=CONICAL_SURFACE ( 'NONE', #123831, 0.1000000000000002554, 0.003490658503988666988 ) ;
#38167=ORIENTED_EDGE ( 'NONE', *, *, #120409, .F. ) ;
#38168=ADVANCED_FACE ( 'NONE', ( #54735 ), #112392, .T. ) ;
#38169=ORIENTED_EDGE ( 'NONE', *, *, #85786, .T. ) ;
#38170=VERTEX_POINT ( 'NONE', #4331 ) ;
#38171=ORIENTED_EDGE ( 'NONE', *, *, #118802, .T. ) ;
#38172=CARTESIAN_POINT ( 'NONE',  ( -10.85000000000000142, 12.50000000000000000, 2.230156782645134950 ) ) ;
#38173=DIRECTION ( 'NONE',  ( -0.000000000000000000, -1.000000000000000000, -0.000000000000000000 ) ) ;
#38174=CARTESIAN_POINT ( 'NONE',  ( -6.650000000000018119, 12.50000000000000000, -2.857883832488653741 ) ) ;
#38175=ORIENTED_EDGE ( 'NONE', *, *, #117149, .F. ) ;
#38176=FACE_BOUND ( 'NONE', #3392, .T. ) ;
#38177=ORIENTED_EDGE ( 'NONE', *, *, #58939, .T. ) ;
#38178=CARTESIAN_POINT ( 'NONE',  ( -13.94999999999998863, 2.500000000000000000, -1.818653347947323917 ) ) ;
#38179=DIRECTION ( 'NONE',  ( 0.000000000000000000, 1.000000000000000000, 0.000000000000000000 ) ) ;
#38180=CIRCLE ( 'NONE', #21446, 0.1000000000000002554 ) ;
#38181=VECTOR ( 'NONE', #39502, 1000.000000000000000 ) ;
#38182=DIRECTION ( 'NONE',  ( 0.000000000000000000, 0.000000000000000000, 1.000000000000000000 ) ) ;
#38183=ADVANCED_FACE ( 'NONE', ( #122851 ), #74593, .T. ) ;
#38184=AXIS2_PLACEMENT_3D ( 'NONE', #8779, #99766, #48736 ) ;
#38185=CARTESIAN_POINT ( 'NONE',  ( 11.24999999999990585, 2.500000000000000000, -5.902370205355750521 ) ) ;
#38186=DIRECTION ( 'NONE',  ( 0.000000000000000000, -0.000000000000000000, 1.000000000000000000 ) ) ;
#38187=FACE_OUTER_BOUND ( 'NONE', #56116, .T. ) ;
#38188=LINE ( 'NONE', #8696, #8101 ) ;
#38189=DIRECTION ( 'NONE',  ( 0.000000000000000000, 0.000000000000000000, 1.000000000000000000 ) ) ;
#38190=EDGE_CURVE ( 'NONE', #93275, #108043, #53476, .T. ) ;
#38191=ADVANCED_FACE ( 'NONE', ( #3711 ), #44279, .T. ) ;
#38192=DIRECTION ( 'NONE',  ( 0.000000000000000000, 1.000000000000000000, 0.000000000000000000 ) ) ;
#38193=EDGE_CURVE ( 'NONE', #127376, #49108, #68324, .T. ) ;
#38194=EDGE_CURVE ( 'NONE', #22334, #43141, #101792, .T. ) ;
#38196=DIRECTION ( 'NONE',  ( 0.000000000000000000, 1.000000000000000000, 0.000000000000000000 ) ) ;
#38197=ORIENTED_EDGE ( 'NONE', *, *, #26388, .T. ) ;
#38198=EDGE_LOOP ( 'NONE', ( #34257, #25157, #66421, #6880 ) ) ;
#38199=ORIENTED_EDGE ( 'NONE', *, *, #9831, .F. ) ;
#38200=VECTOR ( 'NONE', #21638, 1000.000000000000000 ) ;
#38201=EDGE_LOOP ( 'NONE', ( #3553, #22887, #48005, #34159 ) ) ;
#38202=CIRCLE ( 'NONE', #33990, 0.09999999999999982514 ) ;
#38203=AXIS2_PLACEMENT_3D ( 'NONE', #25455, #66678, #106606 ) ;
#38204=DIRECTION ( 'NONE',  ( -0.000000000000000000, -1.000000000000000000, -0.000000000000000000 ) ) ;
#38205=EDGE_CURVE ( 'NONE', #98683, #114600, #26568, .T. ) ;
#38206=DIRECTION ( 'NONE',  ( -0.000000000000000000, 1.000000000000000000, -0.000000000000000000 ) ) ;
#38207=EDGE_CURVE ( 'NONE', #11460, #79421, #18143, .T. ) ;
#38208=ORIENTED_EDGE ( 'NONE', *, *, #49112, .T. ) ;
#38209=VERTEX_POINT ( 'NONE', #12867 ) ;
#38210=ORIENTED_EDGE ( 'NONE', *, *, #30810, .T. ) ;
#38211=DIRECTION ( 'NONE',  ( 0.000000000000000000, -0.9999939076577903929, 0.003490651415223739937 ) ) ;
#38212=EDGE_CURVE ( 'NONE', #113, #11709, #45361, .T. ) ;
#38213=EDGE_CURVE ( 'NONE', #4130, #46755, #91317, .T. ) ;
#38214=DIRECTION ( 'NONE',  ( 0.000000000000000000, 0.000000000000000000, 1.000000000000000000 ) ) ;
#38215=AXIS2_PLACEMENT_3D ( 'NONE', #73264, #5792, #115762 ) ;
#38216=DIRECTION ( 'NONE',  ( -4.274815082592931898E-19, -0.9999939076577903929, -0.003490651415223739937 ) ) ;
#38217=DIRECTION ( 'NONE',  ( 0.000000000000000000, 1.000000000000000000, 0.000000000000000000 ) ) ;
#38218=LINE ( 'NONE', #78142, #72252 ) ;
#38219=DIRECTION ( 'NONE',  ( 0.000000000000000000, 0.000000000000000000, -1.000000000000000000 ) ) ;
#38220=DIRECTION ( 'NONE',  ( -0.000000000000000000, 1.000000000000000000, -0.000000000000000000 ) ) ;
#38221=VERTEX_POINT ( 'NONE', #54108 ) ;
#38222=EDGE_CURVE ( 'NONE', #95448, #117445, #124786, .T. ) ;
#38223=DIRECTION ( 'NONE',  ( 0.000000000000000000, 1.000000000000000000, 0.000000000000000000 ) ) ;
#38224=ORIENTED_EDGE ( 'NONE', *, *, #14902, .T. ) ;
#38225=ORIENTED_EDGE ( 'NONE', *, *, #102731, .F. ) ;
#38226=EDGE_LOOP ( 'NONE', ( #111946, #31572 ) ) ;
#38227=DIRECTION ( 'NONE',  ( 0.000000000000000000, 1.000000000000000000, 0.000000000000000000 ) ) ;
#38228=CIRCLE ( 'NONE', #25687, 0.06509327318403743123 ) ;
#38229=CIRCLE ( 'NONE', #109311, 0.1000000000000002554 ) ;
#38230=ORIENTED_EDGE ( 'NONE', *, *, #84002, .F. ) ;
#38231=ORIENTED_EDGE ( 'NONE', *, *, #100743, .T. ) ;
#38232=DIRECTION ( 'NONE',  ( -0.000000000000000000, 1.000000000000000000, -0.000000000000000000 ) ) ;
#38233=DIRECTION ( 'NONE',  ( 0.000000000000000000, 0.000000000000000000, 1.000000000000000000 ) ) ;
#38234=DIRECTION ( 'NONE',  ( 0.000000000000000000, 1.000000000000000000, 0.000000000000000000 ) ) ;
#38235=CIRCLE ( 'NONE', #6791, 2.000000000000000000 ) ;
#38236=FACE_OUTER_BOUND ( 'NONE', #2243, .T. ) ;
#38237=AXIS2_PLACEMENT_3D ( 'NONE', #126907, #17575, #26768 ) ;
#38238=AXIS2_PLACEMENT_3D ( 'NONE', #105367, #55620, #54332 ) ;
#38239=LINE ( 'NONE', #7461, #97809 ) ;
#38240=EDGE_LOOP ( 'NONE', ( #116775, #1517, #15400, #83695 ) ) ;
#38241=CARTESIAN_POINT ( 'NONE',  ( 1.849999999999950573, 2.500000000000000000, 2.511473670974873507 ) ) ;
#38242=CIRCLE ( 'NONE', #25703, 0.1000000000000002554 ) ;
#38243=AXIS2_PLACEMENT_3D ( 'NONE', #49548, #78364, #88808 ) ;
#38244=ORIENTED_EDGE ( 'NONE', *, *, #57985, .F. ) ;
#38245=DIRECTION ( 'NONE',  ( 0.000000000000000000, 1.000000000000000000, 0.000000000000000000 ) ) ;
#38246=VECTOR ( 'NONE', #50650, 1000.000000000000000 ) ;
#38247=VERTEX_POINT ( 'NONE', #14163 ) ;
#38248=CARTESIAN_POINT ( 'NONE',  ( 12.04999999999990834, 12.50000000000000000, 6.560283801567334372 ) ) ;
#38249=DIRECTION ( 'NONE',  ( -0.000000000000000000, 1.000000000000000000, -0.000000000000000000 ) ) ;
#38250=ORIENTED_EDGE ( 'NONE', *, *, #84587, .F. ) ;
#38251=DIRECTION ( 'NONE',  ( 0.000000000000000000, 0.000000000000000000, 1.000000000000000000 ) ) ;
#38252=DIRECTION ( 'NONE',  ( 0.000000000000000000, 1.000000000000000000, 0.000000000000000000 ) ) ;
#38253=VERTEX_POINT ( 'NONE', #114945 ) ;
#38254=AXIS2_PLACEMENT_3D ( 'NONE', #73021, #110363, #112947 ) ;
#38256=DIRECTION ( 'NONE',  ( -0.000000000000000000, 1.000000000000000000, -0.000000000000000000 ) ) ;
#38257=EDGE_CURVE ( 'NONE', #15629, #92907, #36946, .T. ) ;
#38258=ORIENTED_EDGE ( 'NONE', *, *, #6392, .T. ) ;
#38259=ORIENTED_EDGE ( 'NONE', *, *, #96363, .F. ) ;
#38260=DIRECTION ( 'NONE',  ( 0.000000000000000000, 1.000000000000000000, 0.000000000000000000 ) ) ;
#38263=DIRECTION ( 'NONE',  ( 0.000000000000000000, 1.000000000000000000, 0.000000000000000000 ) ) ;
#38264=VECTOR ( 'NONE', #100429, 1000.000000000000000 ) ;
#38265=FACE_OUTER_BOUND ( 'NONE', #63479, .T. ) ;
#38266=CARTESIAN_POINT ( 'NONE',  ( -3.100000000000028511, 2.500000000000000000, -4.776537180435977525 ) ) ;
#38267=ORIENTED_EDGE ( 'NONE', *, *, #112503, .F. ) ;
#38268=AXIS2_PLACEMENT_3D ( 'NONE', #31097, #100457, #71005 ) ;
#38269=CARTESIAN_POINT ( 'NONE',  ( 87.50000000000001421, 3.975344334345554120, -6.360552532166837914 ) ) ;
#38270=DIRECTION ( 'NONE',  ( 0.000000000000000000, -0.000000000000000000, 1.000000000000000000 ) ) ;
#38271=AXIS2_PLACEMENT_3D ( 'NONE', #24330, #34816, #105468 ) ;
#38272=ORIENTED_EDGE ( 'NONE', *, *, #83556, .F. ) ;
#38273=DIRECTION ( 'NONE',  ( 0.000000000000000000, -0.000000000000000000, 1.000000000000000000 ) ) ;
#38274=DIRECTION ( 'NONE',  ( 0.000000000000000000, -0.000000000000000000, 1.000000000000000000 ) ) ;
#38275=DIRECTION ( 'NONE',  ( 0.000000000000000000, 0.000000000000000000, -1.000000000000000000 ) ) ;
#38276=CARTESIAN_POINT ( 'NONE',  ( -0.2000000000000399791, 12.50000000000000000, -4.676537180435977881 ) ) ;
#38277=AXIS2_PLACEMENT_3D ( 'NONE', #68075, #8498, #58912 ) ;
#38279=AXIS2_PLACEMENT_3D ( 'NONE', #105523, #23745, #14540 ) ;
#38280=ORIENTED_EDGE ( 'NONE', *, *, #110617, .F. ) ;
#38281=CIRCLE ( 'NONE', #21546, 0.06509327318403745899 ) ;
#38282=AXIS2_PLACEMENT_3D ( 'NONE', #64971, #126493, #104895 ) ;
#38283=DIRECTION ( 'NONE',  ( 0.000000000000000000, -0.9999939076577903929, 0.003490651415223739937 ) ) ;
#38284=FACE_OUTER_BOUND ( 'NONE', #124356, .T. ) ;
#38285=AXIS2_PLACEMENT_3D ( 'NONE', #69195, #88176, #98654 ) ;
#38286=ORIENTED_EDGE ( 'NONE', *, *, #11586, .T. ) ;
#38287=DIRECTION ( 'NONE',  ( 0.000000000000000000, 0.000000000000000000, -1.000000000000000000 ) ) ;
#38288=EDGE_CURVE ( 'NONE', #34969, #2954, #51619, .T. ) ;
#38289=EDGE_LOOP ( 'NONE', ( #105775, #44267 ) ) ;
#38290=AXIS2_PLACEMENT_3D ( 'NONE', #9503, #89353, #129301 ) ;
#38291=VECTOR ( 'NONE', #52718, 1000.000000000000000 ) ;
#38292=ORIENTED_EDGE ( 'NONE', *, *, #29884, .T. ) ;
#38293=AXIS2_PLACEMENT_3D ( 'NONE', #9049, #49649, #88235 ) ;
#38294=CARTESIAN_POINT ( 'NONE',  ( 2.949999999999943334, 12.50000000000000000, 6.495190528383297135 ) ) ;
#38295=EDGE_LOOP ( 'NONE', ( #10656, #28480, #80614, #77569 ) ) ;
#38296=CARTESIAN_POINT ( 'NONE',  ( -7.300000000000018474, 12.50000000000000000, -3.983716857408426293 ) ) ;
#38297=DIRECTION ( 'NONE',  ( 0.000000000000000000, 0.000000000000000000, -1.000000000000000000 ) ) ;
#38298=DIRECTION ( 'NONE',  ( 0.000000000000000000, 1.000000000000000000, 0.000000000000000000 ) ) ;
#38299=EDGE_LOOP ( 'NONE', ( #54906, #57785, #54470, #56318 ) ) ;
#38300=LINE ( 'NONE', #48767, #128276 ) ;
#38301=AXIS2_PLACEMENT_3D ( 'NONE', #74404, #94679, #97261 ) ;
#38302=CARTESIAN_POINT ( 'NONE',  ( 4.999999999999935163, 12.50000000000000000, 0.6928203230275494784 ) ) ;
#38303=ORIENTED_EDGE ( 'NONE', *, *, #86182, .T. ) ;
#38304=EDGE_CURVE ( 'NONE', #39786, #25992, #25945, .T. ) ;
#38306=DIRECTION ( 'NONE',  ( 0.000000000000000000, -0.9999939076577903929, 0.003490651415223739937 ) ) ;
#38307=EDGE_CURVE ( 'NONE', #54643, #46118, #118491, .T. ) ;
#38308=ORIENTED_EDGE ( 'NONE', *, *, #64542, .T. ) ;
#38309=ORIENTED_EDGE ( 'NONE', *, *, #93523, .T. ) ;
#38310=EDGE_LOOP ( 'NONE', ( #111007, #40384 ) ) ;
#38311=DIRECTION ( 'NONE',  ( 0.000000000000000000, -0.000000000000000000, 1.000000000000000000 ) ) ;
#38312=FACE_OUTER_BOUND ( 'NONE', #117493, .T. ) ;
#38313=AXIS2_PLACEMENT_3D ( 'NONE', #7131, #87630, #56870 ) ;
#38314=DIRECTION ( 'NONE',  ( 0.000000000000000000, 1.000000000000000000, 0.000000000000000000 ) ) ;
#38315=AXIS2_PLACEMENT_3D ( 'NONE', #56681, #96608, #46896 ) ;
#38316=EDGE_CURVE ( 'NONE', #32403, #80982, #95963, .T. ) ;
#38317=FACE_BOUND ( 'NONE', #107564, .T. ) ;
#38318=ORIENTED_EDGE ( 'NONE', *, *, #43732, .T. ) ;
#38320=CARTESIAN_POINT ( 'NONE',  ( 1.449999999999952216, 2.500000000000000000, -2.411473670974877859 ) ) ;
#38321=EDGE_LOOP ( 'NONE', ( #25648, #13398 ) ) ;
#38323=AXIS2_PLACEMENT_3D ( 'NONE', #38294, #117446, #78221 ) ;
#38324=CARTESIAN_POINT ( 'NONE',  ( 6.449999999999931788, 12.50000000000000000, -6.148780366869526226 ) ) ;
#38325=AXIS2_PLACEMENT_3D ( 'NONE', #48462, #59604, #28184 ) ;
#38326=AXIS2_PLACEMENT_3D ( 'NONE', #7108, #16274, #94862 ) ;
#38327=DIRECTION ( 'NONE',  ( 0.000000000000000000, 1.000000000000000000, 0.000000000000000000 ) ) ;
#38328=CIRCLE ( 'NONE', #55032, 0.09999999999999982514 ) ;
#38329=DIRECTION ( 'NONE',  ( 0.000000000000000000, -0.000000000000000000, 1.000000000000000000 ) ) ;
#38330=CARTESIAN_POINT ( 'NONE',  ( 5.449999999999936229, 12.50000000000000000, -2.099970236277064473 ) ) ;
#38331=DIRECTION ( 'NONE',  ( 0.000000000000000000, 0.000000000000000000, -1.000000000000000000 ) ) ;
#38332=CARTESIAN_POINT ( 'NONE',  ( -5.800000000000018474, 12.50000000000000000, 4.395220292106234439 ) ) ;
#38333=AXIS2_PLACEMENT_3D ( 'NONE', #31505, #51799, #71408 ) ;
#38334=AXIS2_PLACEMENT_3D ( 'NONE', #61940, #101856, #12165 ) ;
#38335=AXIS2_PLACEMENT_3D ( 'NONE', #21187, #61113, #101042 ) ;
#38336=ORIENTED_EDGE ( 'NONE', *, *, #77191, .F. ) ;
#38337=VERTEX_POINT ( 'NONE', #125428 ) ;
#38338=VERTEX_POINT ( 'NONE', #7569 ) ;
#38339=ORIENTED_EDGE ( 'NONE', *, *, #21012, .F. ) ;
#38340=CIRCLE ( 'NONE', #55047, 0.1000000000000002554 ) ;
#38341=ORIENTED_EDGE ( 'NONE', *, *, #22400, .F. ) ;
#38342=DIRECTION ( 'NONE',  ( 0.000000000000000000, 0.000000000000000000, 1.000000000000000000 ) ) ;
#38343=PLANE ( 'NONE',  #15370 ) ;
#38344=ORIENTED_EDGE ( 'NONE', *, *, #48389, .F. ) ;
#38345=FACE_BOUND ( 'NONE', #4748, .T. ) ;
#38346=CARTESIAN_POINT ( 'NONE',  ( -13.74999999999998934, 2.500000000000000000, -1.572243186433547990 ) ) ;
#38347=ADVANCED_FACE ( 'NONE', ( #108358 ), #87097, .T. ) ;
#38348=DIRECTION ( 'NONE',  ( -0.000000000000000000, -1.000000000000000000, -0.000000000000000000 ) ) ;
#38349=CARTESIAN_POINT ( 'NONE',  ( -2.900000000000029221, 12.50000000000000000, -5.022947341949754119 ) ) ;
#38351=LINE ( 'NONE', #59290, #101419 ) ;
#38352=EDGE_CURVE ( 'NONE', #34182, #52632, #35760, .T. ) ;
#38353=CARTESIAN_POINT ( 'NONE',  ( -13.34999999999999076, 12.50000000000000000, 1.472243186433549456 ) ) ;
#38354=VERTEX_POINT ( 'NONE', #6272 ) ;
#38355=LINE ( 'NONE', #40785, #72384 ) ;
#38356=ADVANCED_FACE ( 'NONE', ( #116240 ), #95527, .T. ) ;
#38357=VECTOR ( 'NONE', #112185, 1000.000000000000000 ) ;
#38358=ORIENTED_EDGE ( 'NONE', *, *, #66721, .T. ) ;
#38359=ORIENTED_EDGE ( 'NONE', *, *, #46976, .T. ) ;
#38360=ORIENTED_EDGE ( 'NONE', *, *, #85868, .F. ) ;
#38361=EDGE_CURVE ( 'NONE', #99244, #68489, #112255, .T. ) ;
#38362=CARTESIAN_POINT ( 'NONE',  ( 12.94999999999990337, 12.50000000000000000, 2.165063509461097713 ) ) ;
#38363=DIRECTION ( 'NONE',  ( 0.000000000000000000, 1.000000000000000000, 0.000000000000000000 ) ) ;
#38364=ADVANCED_FACE ( 'NONE', ( #46217 ), #6909, .T. ) ;
#38365=DIRECTION ( 'NONE',  ( 0.000000000000000000, 0.000000000000000000, -1.000000000000000000 ) ) ;
#38366=EDGE_CURVE ( 'NONE', #22212, #101321, #55810, .T. ) ;
#38368=DIRECTION ( 'NONE',  ( 0.000000000000000000, -0.9999939076577903929, 0.003490651415223739937 ) ) ;
#38369=EDGE_CURVE ( 'NONE', #51769, #57444, #3581, .T. ) ;
#38370=CIRCLE ( 'NONE', #69647, 0.06509327318403745899 ) ;
#38371=VECTOR ( 'NONE', #47993, 1000.000000000000000 ) ;
#38372=VECTOR ( 'NONE', #82252, 1000.000000000000000 ) ;
#38373=DIRECTION ( 'NONE',  ( 0.000000000000000000, 0.000000000000000000, 1.000000000000000000 ) ) ;
#38374=DIRECTION ( 'NONE',  ( 0.000000000000000000, 1.000000000000000000, 0.000000000000000000 ) ) ;
#38375=ADVANCED_FACE ( 'NONE', ( #116874 ), #5635, .T. ) ;
#38377=CARTESIAN_POINT ( 'NONE',  ( 12.69999999999989804, 2.500000000000000000, 0.2464101615137735679 ) ) ;
#38378=CARTESIAN_POINT ( 'NONE',  ( 0.000000000000000000, 2.500000000000000000, 0.000000000000000000 ) ) ;
#38379=PLANE ( 'NONE',  #85083 ) ;
#38380=CIRCLE ( 'NONE', #88517, 0.06509327318403745899 ) ;
#38381=ORIENTED_EDGE ( 'NONE', *, *, #42794, .T. ) ;
#38382=CARTESIAN_POINT ( 'NONE',  ( -9.550000000000007816, 12.50000000000000000, -6.430097255199259010 ) ) ;
#38383=CIRCLE ( 'NONE', #63405, 0.06509327318403745899 ) ;
#38384=ADVANCED_FACE ( 'NONE', ( #86118 ), #116436, .T. ) ;
#38385=CIRCLE ( 'NONE', #82287, 0.1000000000000002554 ) ;
#38387=CIRCLE ( 'NONE', #53042, 0.06509327318403745899 ) ;
#38388=ORIENTED_EDGE ( 'NONE', *, *, #41476, .T. ) ;
#38389=CARTESIAN_POINT ( 'NONE',  ( 4.149999999999938183, 2.500000000000000000, 5.902370205355745192 ) ) ;
#38390=CARTESIAN_POINT ( 'NONE',  ( 8.349999999999919709, 12.50000000000000000, 5.737276932171707422 ) ) ;
#38391=DIRECTION ( 'NONE',  ( -0.000000000000000000, 1.000000000000000000, -0.000000000000000000 ) ) ;
#38392=AXIS2_PLACEMENT_3D ( 'NONE', #43044, #39958, #13540 ) ;
#38394=ORIENTED_EDGE ( 'NONE', *, *, #127581, .F. ) ;
#38395=DIRECTION ( 'NONE',  ( -0.000000000000000000, 1.000000000000000000, -0.000000000000000000 ) ) ;
#38396=DIRECTION ( 'NONE',  ( 0.000000000000000000, 0.000000000000000000, -1.000000000000000000 ) ) ;
#38397=VECTOR ( 'NONE', #109619, 1000.000000000000000 ) ;
#38398=CONICAL_SURFACE ( 'NONE', #111531, 0.09999999999999982514, 0.003490658503988666988 ) ;
#38399=AXIS2_PLACEMENT_3D ( 'NONE', #74433, #35791, #3746 ) ;
#38400=CARTESIAN_POINT ( 'NONE',  ( -7.300000000000013145, 2.500000000000000000, 3.983716857408420076 ) ) ;
#38401=ORIENTED_EDGE ( 'NONE', *, *, #104007, .T. ) ;
#38402=ORIENTED_EDGE ( 'NONE', *, *, #99348, .F. ) ;
#38403=CARTESIAN_POINT ( 'NONE',  ( 1.849999999999949685, 12.50000000000000000, -2.576566944158915184 ) ) ;
#38404=CIRCLE ( 'NONE', #34193, 0.06509327318403745899 ) ;
#38405=ORIENTED_EDGE ( 'NONE', *, *, #45021, .F. ) ;
#38406=AXIS2_PLACEMENT_3D ( 'NONE', #112077, #61033, #111407 ) ;
#38407=CARTESIAN_POINT ( 'NONE',  ( 6.649999999999928413, 2.500000000000000000, 2.957883832488649389 ) ) ;
#38408=DIRECTION ( 'NONE',  ( 0.000000000000000000, -0.000000000000000000, 1.000000000000000000 ) ) ;
#38409=VERTEX_POINT ( 'NONE', #45588 ) ;
#38410=DIRECTION ( 'NONE',  ( 0.000000000000000000, 0.000000000000000000, 1.000000000000000000 ) ) ;
#38411=CARTESIAN_POINT ( 'NONE',  ( -11.89999999999999680, 2.500000000000000000, -0.3464101615137741841 ) ) ;
#38413=CARTESIAN_POINT ( 'NONE',  ( -1.650000000000034772, 2.500000000000000000, 6.495190528383297135 ) ) ;
#38414=ORIENTED_EDGE ( 'NONE', *, *, #50966, .T. ) ;
#38415=CARTESIAN_POINT ( 'NONE',  ( -7.500000000000016875, 2.500000000000000000, 0.6928203230275494784 ) ) ;
#38416=ADVANCED_FACE ( 'NONE', ( #126058 ), #67111, .T. ) ;
#38417=ORIENTED_EDGE ( 'NONE', *, *, #71786, .T. ) ;
#38418=ORIENTED_EDGE ( 'NONE', *, *, #69846, .F. ) ;
#38419=CIRCLE ( 'NONE', #11294, 0.06509327318403745899 ) ;
#38420=CIRCLE ( 'NONE', #59351, 0.1000000000000002554 ) ;
#38421=DIRECTION ( 'NONE',  ( 0.000000000000000000, 1.000000000000000000, 0.000000000000000000 ) ) ;
#38422=DIRECTION ( 'NONE',  ( -0.000000000000000000, 1.000000000000000000, -0.000000000000000000 ) ) ;
#38423=FACE_OUTER_BOUND ( 'NONE', #97391, .T. ) ;
#38424=DIRECTION ( 'NONE',  ( 0.000000000000000000, -0.9999939076577903929, 0.003490651415223739937 ) ) ;
#38425=CARTESIAN_POINT ( 'NONE',  ( -14.79999999999998295, 12.50000000000000000, -0.3464101615137760715 ) ) ;
#38426=DIRECTION ( 'NONE',  ( 0.000000000000000000, 0.000000000000000000, 1.000000000000000000 ) ) ;
#38427=EDGE_CURVE ( 'NONE', #49328, #21207, #7670, .T. ) ;
#38428=AXIS2_PLACEMENT_3D ( 'NONE', #69672, #109611, #10114 ) ;
#38429=CARTESIAN_POINT ( 'NONE',  ( -0.6500000000000403233, 2.500000000000000000, 1.918653347947321564 ) ) ;
#38430=CONICAL_SURFACE ( 'NONE', #88577, 0.1000000000000002554, 0.003490658503988666988 ) ;
#38431=DIRECTION ( 'NONE',  ( 0.000000000000000000, -0.9999939076577903929, 0.003490651415223739937 ) ) ;
#38432=DIRECTION ( 'NONE',  ( 0.000000000000000000, -0.9999939076577903929, 0.003490651415223739937 ) ) ;
#38433=VECTOR ( 'NONE', #53868, 1000.000000000000000 ) ;
#38434=DIRECTION ( 'NONE',  ( 0.000000000000000000, 0.000000000000000000, 1.000000000000000000 ) ) ;
#38435=CIRCLE ( 'NONE', #113731, 0.06509327318403745899 ) ;
#38436=CIRCLE ( 'NONE', #94845, 0.09999999999999999167 ) ;
#38437=AXIS2_PLACEMENT_3D ( 'NONE', #67599, #8038, #107543 ) ;
#38438=VERTEX_POINT ( 'NONE', #97251 ) ;
#38439=PLANE ( 'NONE',  #84236 ) ;
#38440=DIRECTION ( 'NONE',  ( -0.000000000000000000, -1.000000000000000000, -0.000000000000000000 ) ) ;
#38441=FACE_OUTER_BOUND ( 'NONE', #64951, .T. ) ;
#38443=FACE_OUTER_BOUND ( 'NONE', #104548, .T. ) ;
#38444=ORIENTED_EDGE ( 'NONE', *, *, #83133, .T. ) ;
#38445=DIRECTION ( 'NONE',  ( 0.000000000000000000, 0.000000000000000000, -1.000000000000000000 ) ) ;
#38447=LINE ( 'NONE', #128769, #73502 ) ;
#38448=ORIENTED_EDGE ( 'NONE', *, *, #20447, .T. ) ;
#38449=AXIS2_PLACEMENT_3D ( 'NONE', #23008, #62296, #102215 ) ;
#38450=ORIENTED_EDGE ( 'NONE', *, *, #90511, .F. ) ;
#38451=CARTESIAN_POINT ( 'NONE',  ( -6.900000000000019007, 12.50000000000000000, -3.983716857408426293 ) ) ;
#38453=ORIENTED_EDGE ( 'NONE', *, *, #41465, .F. ) ;
#38454=ORIENTED_EDGE ( 'NONE', *, *, #114417, .T. ) ;
#38455=EDGE_LOOP ( 'NONE', ( #108958, #128699 ) ) ;
#38456=CARTESIAN_POINT ( 'NONE',  ( 4.149999999999938183, 2.500000000000000000, 2.065063509461097624 ) ) ;
#38457=CARTESIAN_POINT ( 'NONE',  ( 0.6499999999999561684, 12.50000000000000000, -1.753560074763288457 ) ) ;
#38458=DIRECTION ( 'NONE',  ( 0.000000000000000000, 1.000000000000000000, 0.000000000000000000 ) ) ;
#38460=DIRECTION ( 'NONE',  ( -0.000000000000000000, 1.000000000000000000, -0.000000000000000000 ) ) ;
#38461=ADVANCED_FACE ( 'NONE', ( #71661 ), #80949, .T. ) ;
#38462=AXIS2_PLACEMENT_3D ( 'NONE', #125070, #76619, #85777 ) ;
#38463=ORIENTED_EDGE ( 'NONE', *, *, #112053, .T. ) ;
#38464=CARTESIAN_POINT ( 'NONE',  ( 9.599999999999914380, 2.500000000000000000, 4.330127018922196314 ) ) ;
#38465=ORIENTED_EDGE ( 'NONE', *, *, #93932, .F. ) ;
#38466=PLANE ( 'NONE',  #62231 ) ;
#38467=CARTESIAN_POINT ( 'NONE',  ( 6.449999999999931788, 2.500000000000000000, -6.148780366869526226 ) ) ;
#38468=EDGE_CURVE ( 'NONE', #20444, #13136, #62177, .T. ) ;
#38469=CARTESIAN_POINT ( 'NONE',  ( 18.37149739119579905, 2.540880845002019495, 2.596776292459959112 ) ) ;
#38470=PLANE ( 'NONE',  #75622 ) ;
#38471=DIRECTION ( 'NONE',  ( -4.274815082592931898E-19, -0.9999939076577903929, -0.003490651415223739937 ) ) ;
#38472=CONICAL_SURFACE ( 'NONE', #111610, 0.1000000000000000472, 0.003490658503988666988 ) ;
#38473=EDGE_CURVE ( 'NONE', #79548, #87068, #111587, .T. ) ;
#38474=CONICAL_SURFACE ( 'NONE', #126187, 0.1000000000000000472, 0.003490658503988666988 ) ;
#38475=CONICAL_SURFACE ( 'NONE', #111614, 0.09999999999999999167, 0.003490658503988666988 ) ;
#38476=ORIENTED_EDGE ( 'NONE', *, *, #126956, .F. ) ;
#38477=VECTOR ( 'NONE', #120856, 1000.000000000000000 ) ;
#38478=ORIENTED_EDGE ( 'NONE', *, *, #60804, .F. ) ;
#38479=EDGE_CURVE ( 'NONE', #16041, #128284, #89356, .T. ) ;
#38480=EDGE_LOOP ( 'NONE', ( #40107, #42324, #73795, #96454 ) ) ;
#38481=ORIENTED_EDGE ( 'NONE', *, *, #43334, .F. ) ;
#38482=EDGE_LOOP ( 'NONE', ( #122900, #29515 ) ) ;
#38483=FACE_OUTER_BOUND ( 'NONE', #41780, .T. ) ;
#38484=DIRECTION ( 'NONE',  ( -0.000000000000000000, -1.000000000000000000, -0.000000000000000000 ) ) ;
#38485=DIRECTION ( 'NONE',  ( -0.000000000000000000, -1.000000000000000000, -0.000000000000000000 ) ) ;
#38486=ADVANCED_FACE ( 'NONE', ( #99848 ), #106075, .T. ) ;
#38487=FACE_BOUND ( 'NONE', #39878, .T. ) ;
#38488=DIRECTION ( 'NONE',  ( 0.000000000000000000, -0.000000000000000000, 1.000000000000000000 ) ) ;
#38489=DIRECTION ( 'NONE',  ( -0.000000000000000000, 1.000000000000000000, -0.000000000000000000 ) ) ;
#38490=PLANE ( 'NONE',  #69872 ) ;
#38491=PLANE ( 'NONE',  #87654 ) ;
#38492=AXIS2_PLACEMENT_3D ( 'NONE', #114751, #75473, #66930 ) ;
#38493=CONICAL_SURFACE ( 'NONE', #53054, 0.09999999999999982514, 0.003490658503988666988 ) ;
#38494=AXIS2_PLACEMENT_3D ( 'NONE', #19119, #40081, #78063 ) ;
#38496=CARTESIAN_POINT ( 'NONE',  ( -9.150000000000009237, 12.50000000000000000, 2.857883832488649301 ) ) ;
#38497=AXIS2_PLACEMENT_3D ( 'NONE', #29641, #40112, #57163 ) ;
#38498=DIRECTION ( 'NONE',  ( 0.000000000000000000, 1.000000000000000000, 0.000000000000000000 ) ) ;
#38499=AXIS2_PLACEMENT_3D ( 'NONE', #1747, #82265, #2376 ) ;
#38500=CARTESIAN_POINT ( 'NONE',  ( -12.89999999999999147, 12.50000000000000000, -0.06509327318403558549 ) ) ;
#38501=ORIENTED_EDGE ( 'NONE', *, *, #20882, .T. ) ;
#38502=EDGE_LOOP ( 'NONE', ( #103723, #1242 ) ) ;
#38503=VERTEX_POINT ( 'NONE', #120125 ) ;
#38504=ORIENTED_EDGE ( 'NONE', *, *, #100524, .T. ) ;
#38505=DIRECTION ( 'NONE',  ( -0.000000000000000000, -1.000000000000000000, -0.000000000000000000 ) ) ;
#38506=FACE_BOUND ( 'NONE', #53234, .T. ) ;
#38507=CARTESIAN_POINT ( 'NONE',  ( 5.649999999999934630, 2.500000000000000000, -2.511473670974877948 ) ) ;
#38508=VECTOR ( 'NONE', #110518, 1000.000000000000000 ) ;
#38509=AXIS2_PLACEMENT_3D ( 'NONE', #39712, #99258, #48872 ) ;
#38510=VERTEX_POINT ( 'NONE', #108989 ) ;
#38511=CARTESIAN_POINT ( 'NONE',  ( 5.849999999999932143, 2.500000000000000000, 1.472243186433545459 ) ) ;
#38512=AXIS2_PLACEMENT_3D ( 'NONE', #109825, #20155, #82310 ) ;
#38513=DIRECTION ( 'NONE',  ( 0.000000000000000000, -0.9999939076577903929, 0.003490651415223739937 ) ) ;
#38514=CARTESIAN_POINT ( 'NONE',  ( 10.84999999999990905, 2.500000000000000000, -5.802370205355749988 ) ) ;
#38515=DIRECTION ( 'NONE',  ( 0.000000000000000000, 0.000000000000000000, 1.000000000000000000 ) ) ;
#38516=EDGE_LOOP ( 'NONE', ( #84195, #122682 ) ) ;
#38517=CARTESIAN_POINT ( 'NONE',  ( 18.09027855933890550, 2.526462839860865284, -2.685672775344708718 ) ) ;
#38518=EDGE_CURVE ( 'NONE', #14289, #39788, #20305, .T. ) ;
#38519=AXIS2_PLACEMENT_3D ( 'NONE', #35055, #62575, #74959 ) ;
#38520=VECTOR ( 'NONE', #38944, 1000.000000000000000 ) ;
#38521=ORIENTED_EDGE ( 'NONE', *, *, #63037, .F. ) ;
#38522=EDGE_CURVE ( 'NONE', #52139, #34976, #24515, .T. ) ;
#38523=EDGE_LOOP ( 'NONE', ( #30061, #12707 ) ) ;
#38524=EDGE_CURVE ( 'NONE', #62921, #86305, #29809, .T. ) ;
#38525=CARTESIAN_POINT ( 'NONE',  ( 5.649999999999932854, 2.500000000000000000, 2.511473670974873507 ) ) ;
#38526=PLANE ( 'NONE',  #102006 ) ;
#38527=ADVANCED_FACE ( 'NONE', ( #19322 ), #69730, .T. ) ;
#38528=EDGE_LOOP ( 'NONE', ( #97212, #18867 ) ) ;
#38529=ADVANCED_FACE ( 'NONE', ( #319 ), #129323, .T. ) ;
#38530=AXIS2_PLACEMENT_3D ( 'NONE', #121019, #90916, #41197 ) ;
#38531=CIRCLE ( 'NONE', #105408, 0.06509327318403745899 ) ;
#38532=CARTESIAN_POINT ( 'NONE',  ( -14.59999999999998366, 2.500000000000000000, -0.5928203230275519431 ) ) ;
#38533=DIRECTION ( 'NONE',  ( 0.000000000000000000, -0.9999939076577903929, 0.003490651415223739937 ) ) ;
#38534=ORIENTED_EDGE ( 'NONE', *, *, #16877, .T. ) ;
#38535=CARTESIAN_POINT ( 'NONE',  ( -5.850000000000018296, 2.500000000000000000, 1.472243186433545459 ) ) ;
#38536=EDGE_CURVE ( 'NONE', #53623, #72821, #70374, .T. ) ;
#38537=AXIS2_PLACEMENT_3D ( 'NONE', #98116, #106652, #115829 ) ;
#38538=ORIENTED_EDGE ( 'NONE', *, *, #82559, .T. ) ;
#38539=FACE_OUTER_BOUND ( 'NONE', #41035, .T. ) ;
#38540=ORIENTED_EDGE ( 'NONE', *, *, #80290, .F. ) ;
#38541=DIRECTION ( 'NONE',  ( -0.000000000000000000, -1.000000000000000000, -0.000000000000000000 ) ) ;
#38542=FACE_BOUND ( 'NONE', #70103, .T. ) ;
#38543=EDGE_CURVE ( 'NONE', #18013, #32951, #85134, .T. ) ;
#38544=ADVANCED_FACE ( 'NONE', ( #49468 ), #91399, .T. ) ;
#38545=EDGE_LOOP ( 'NONE', ( #3228, #95436, #104975, #25242 ) ) ;
#38546=CARTESIAN_POINT ( 'NONE',  ( 5.849999999999934808, 12.50000000000000000, -5.737276932171712751 ) ) ;
#38547=EDGE_LOOP ( 'NONE', ( #59247, #399, #113525, #20976 ) ) ;
#38548=DIRECTION ( 'NONE',  ( 0.000000000000000000, 0.000000000000000000, 1.000000000000000000 ) ) ;
#38549=LINE ( 'NONE', #28060, #123986 ) ;
#38550=FACE_OUTER_BOUND ( 'NONE', #125917, .T. ) ;
#38551=CARTESIAN_POINT ( 'NONE',  ( -10.20000000000000639, 2.500000000000000000, -3.983716857408421852 ) ) ;
#38552=CARTESIAN_POINT ( 'NONE',  ( 17.50000000000000355, 2.413248583741727682, -3.595440551767597359 ) ) ;
#38553=EDGE_LOOP ( 'NONE', ( #1896, #79302 ) ) ;
#38554=ORIENTED_EDGE ( 'NONE', *, *, #74097, .F. ) ;
#38555=ORIENTED_EDGE ( 'NONE', *, *, #60912, .F. ) ;
#38556=FACE_OUTER_BOUND ( 'NONE', #111898, .T. ) ;
#38557=CARTESIAN_POINT ( 'NONE',  ( 11.64999999999990621, 2.500000000000000000, 6.595190528383296780 ) ) ;
#38558=CARTESIAN_POINT ( 'NONE',  ( 3.099999999999945022, 2.500000000000000000, -0.4464101615137783252 ) ) ;
#38559=ORIENTED_EDGE ( 'NONE', *, *, #71565, .T. ) ;
#38560=ORIENTED_EDGE ( 'NONE', *, *, #118102, .T. ) ;
#38561=EDGE_LOOP ( 'NONE', ( #88918, #5885 ) ) ;
#38562=LINE ( 'NONE', #60132, #35212 ) ;
#38563=CIRCLE ( 'NONE', #65623, 0.06509327318403741736 ) ;
#38564=PLANE ( 'NONE',  #115483 ) ;
#38565=VECTOR ( 'NONE', #40590, 1000.000000000000000 ) ;
#38567=FACE_OUTER_BOUND ( 'NONE', #68785, .T. ) ;
#38568=FACE_OUTER_BOUND ( 'NONE', #12672, .T. ) ;
#38569=CARTESIAN_POINT ( 'NONE',  ( 7.949999999999925571, 2.500000000000000000, -6.595190528383302109 ) ) ;
#38570=CARTESIAN_POINT ( 'NONE',  ( -12.49999999999999467, 12.50000000000000000, -3.702399969078684627 ) ) ;
#38573=EDGE_LOOP ( 'NONE', ( #95881, #80814 ) ) ;
#38574=ORIENTED_EDGE ( 'NONE', *, *, #1295, .T. ) ;
#38575=AXIS2_PLACEMENT_3D ( 'NONE', #8799, #76272, #116824 ) ;
#38576=DIRECTION ( 'NONE',  ( 0.000000000000000000, 0.000000000000000000, -1.000000000000000000 ) ) ;
#38577=LINE ( 'NONE', #28743, #57051 ) ;
#38578=VERTEX_POINT ( 'NONE', #41585 ) ;
#38579=EDGE_LOOP ( 'NONE', ( #127153, #92468, #27256, #23442 ) ) ;
#38581=CARTESIAN_POINT ( 'NONE',  ( -4.800000000000022915, 12.50000000000000000, 3.983716857408420076 ) ) ;
#38582=DIRECTION ( 'NONE',  ( 0.000000000000000000, 1.000000000000000000, 0.000000000000000000 ) ) ;
#38583=DIRECTION ( 'NONE',  ( 0.000000000000000000, 0.000000000000000000, 1.000000000000000000 ) ) ;
#38584=EDGE_CURVE ( 'NONE', #82532, #51256, #47501, .T. ) ;
#38585=AXIS2_PLACEMENT_3D ( 'NONE', #56319, #26236, #5915 ) ;
#38586=DIRECTION ( 'NONE',  ( 0.000000000000000000, 0.000000000000000000, -1.000000000000000000 ) ) ;
#38587=VECTOR ( 'NONE', #67110, 1000.000000000000000 ) ;
#38588=CARTESIAN_POINT ( 'NONE',  ( 14.34999999999989662, 12.50000000000000000, 1.753560074763284016 ) ) ;
#38589=DIRECTION ( 'NONE',  ( 0.000000000000000000, 0.000000000000000000, -1.000000000000000000 ) ) ;
#38590=CIRCLE ( 'NONE', #122196, 0.06509327318403745899 ) ;
#38591=AXIS2_PLACEMENT_3D ( 'NONE', #106398, #73706, #55375 ) ;
#38592=FACE_OUTER_BOUND ( 'NONE', #29511, .T. ) ;
#38593=VERTEX_POINT ( 'NONE', #59289 ) ;
#38594=ORIENTED_EDGE ( 'NONE', *, *, #113141, .F. ) ;
#38595=ORIENTED_EDGE ( 'NONE', *, *, #123882, .F. ) ;
#38596=VERTEX_POINT ( 'NONE', #40943 ) ;
#38597=CARTESIAN_POINT ( 'NONE',  ( 13.74999999999989875, 12.50000000000000000, 1.472243186433545459 ) ) ;
#38598=CARTESIAN_POINT ( 'NONE',  ( 1.249999999999950262, 12.50000000000000000, 7.122917578226811486 ) ) ;
#38599=EDGE_LOOP ( 'NONE', ( #89384, #97238, #11562, #1021 ) ) ;
#38600=LINE ( 'NONE', #70615, #36080 ) ;
#38601=DIRECTION ( 'NONE',  ( -0.000000000000000000, -1.000000000000000000, -0.000000000000000000 ) ) ;
#38602=VECTOR ( 'NONE', #50459, 1000.000000000000000 ) ;
#38603=AXIS2_PLACEMENT_3D ( 'NONE', #118249, #79616, #69138 ) ;
#38604=DIRECTION ( 'NONE',  ( -0.000000000000000000, 1.000000000000000000, -0.000000000000000000 ) ) ;
#38605=DIRECTION ( 'NONE',  ( 0.000000000000000000, 0.000000000000000000, 1.000000000000000000 ) ) ;
#38606=EDGE_LOOP ( 'NONE', ( #34021, #106470, #46297, #97542 ) ) ;
#38607=AXIS2_PLACEMENT_3D ( 'NONE', #44845, #104399, #54637 ) ;
#38608=CIRCLE ( 'NONE', #128485, 0.06509327318403745899 ) ;
#38609=CARTESIAN_POINT ( 'NONE',  ( -7.050000000000013145, 12.50000000000000000, 6.560283801567334372 ) ) ;
#38610=DIRECTION ( 'NONE',  ( 0.000000000000000000, 0.000000000000000000, 1.000000000000000000 ) ) ;
#38611=ORIENTED_EDGE ( 'NONE', *, *, #4144, .F. ) ;
#38612=CONICAL_SURFACE ( 'NONE', #69894, 0.1000000000000000472, 0.003490658503988666988 ) ;
#38613=AXIS2_PLACEMENT_3D ( 'NONE', #64892, #104808, #124477 ) ;
#38614=CIRCLE ( 'NONE', #78414, 0.06509327318403745899 ) ;
#38615=ORIENTED_EDGE ( 'NONE', *, *, #21917, .F. ) ;
#38616=ORIENTED_EDGE ( 'NONE', *, *, #38207, .F. ) ;
#38617=CARTESIAN_POINT ( 'NONE',  ( -11.24999999999999822, 12.50000000000000000, 1.472243186433545459 ) ) ;
#38618=AXIS2_PLACEMENT_3D ( 'NONE', #87031, #67359, #126967 ) ;
#38620=AXIS2_PLACEMENT_3D ( 'NONE', #57559, #7797, #97473 ) ;
#38621=AXIS2_PLACEMENT_3D ( 'NONE', #63446, #103372, #70685 ) ;
#38622=ADVANCED_FACE ( 'NONE', ( #99201 ), #49665, .T. ) ;
#38623=CIRCLE ( 'NONE', #36568, 0.1000000000000002554 ) ;
#38624=VERTEX_POINT ( 'NONE', #89378 ) ;
#38626=DIRECTION ( 'NONE',  ( -0.000000000000000000, -1.000000000000000000, -0.000000000000000000 ) ) ;
#38627=EDGE_CURVE ( 'NONE', #122449, #46062, #39210, .T. ) ;
#38628=DIRECTION ( 'NONE',  ( -4.274815082592931898E-19, -0.9999939076577903929, -0.003490651415223739937 ) ) ;
#38629=DIRECTION ( 'NONE',  ( -0.000000000000000000, -1.000000000000000000, -0.000000000000000000 ) ) ;
#38630=EDGE_CURVE ( 'NONE', #66522, #53654, #108126, .T. ) ;
#38631=EDGE_LOOP ( 'NONE', ( #66924, #7163 ) ) ;
#38632=DIRECTION ( 'NONE',  ( 0.000000000000000000, 0.000000000000000000, 1.000000000000000000 ) ) ;
#38633=ORIENTED_EDGE ( 'NONE', *, *, #83144, .F. ) ;
#38634=ADVANCED_FACE ( 'NONE', ( #54580 ), #94515, .T. ) ;
#38636=ORIENTED_EDGE ( 'NONE', *, *, #32181, .F. ) ;
#38637=PLANE ( 'NONE',  #72973 ) ;
#38638=EDGE_CURVE ( 'NONE', #75229, #85897, #124862, .T. ) ;
#38639=DIRECTION ( 'NONE',  ( 0.000000000000000000, -0.000000000000000000, 1.000000000000000000 ) ) ;
#38640=EDGE_CURVE ( 'NONE', #16894, #76479, #60133, .T. ) ;
#38641=FACE_BOUND ( 'NONE', #124560, .T. ) ;
#38642=CARTESIAN_POINT ( 'NONE',  ( -3.150000000000030109, 2.500000000000000000, 1.718653347947321386 ) ) ;
#38643=CIRCLE ( 'NONE', #69921, 0.1000000000000000056 ) ;
#38644=DIRECTION ( 'NONE',  ( 0.000000000000000000, 0.000000000000000000, 1.000000000000000000 ) ) ;
#38645=FACE_OUTER_BOUND ( 'NONE', #31608, .T. ) ;
#38646=VERTEX_POINT ( 'NONE', #52035 ) ;
#38647=FACE_OUTER_BOUND ( 'NONE', #107100, .T. ) ;
#38648=DIRECTION ( 'NONE',  ( 0.000000000000000000, -0.9999939076577903929, 0.003490651415223739937 ) ) ;
#38649=ADVANCED_FACE ( 'NONE', ( #123343 ), #112337, .T. ) ;
#38650=CARTESIAN_POINT ( 'NONE',  ( 12.49999999999990408, 12.50000000000000000, 5.022947341949748790 ) ) ;
#38651=CARTESIAN_POINT ( 'NONE',  ( -0.6500000000000403233, 12.50000000000000000, 1.818653347947321475 ) ) ;
#38652=VERTEX_POINT ( 'NONE', #82128 ) ;
#38653=CONICAL_SURFACE ( 'NONE', #44896, 0.1000000000000002554, 0.003490658503988666988 ) ;
#38654=AXIS2_PLACEMENT_3D ( 'NONE', #29948, #58760, #88860 ) ;
#38656=DIRECTION ( 'NONE',  ( -0.000000000000000000, -1.000000000000000000, -0.000000000000000000 ) ) ;
#38657=EDGE_LOOP ( 'NONE', ( #40508, #34558, #98773, #89133 ) ) ;
#38658=ORIENTED_EDGE ( 'NONE', *, *, #75847, .T. ) ;
#38659=LINE ( 'NONE', #58920, #83634 ) ;
#38660=CARTESIAN_POINT ( 'NONE',  ( 3.149999999999946176, 2.500000000000000000, -6.048780366869526581 ) ) ;
#38661=FACE_BOUND ( 'NONE', #106981, .T. ) ;
#38662=CARTESIAN_POINT ( 'NONE',  ( 13.39473262249371999, -2.500000000000000000, -7.044698190877974220 ) ) ;
#38663=ORIENTED_EDGE ( 'NONE', *, *, #103174, .F. ) ;
#38664=DIRECTION ( 'NONE',  ( -0.000000000000000000, -1.000000000000000000, -0.000000000000000000 ) ) ;
#38665=CONICAL_SURFACE ( 'NONE', #26035, 0.1000000000000002554, 0.003490658503988666988 ) ;
#38666=ORIENTED_EDGE ( 'NONE', *, *, #60516, .T. ) ;
#38667=VERTEX_POINT ( 'NONE', #113514 ) ;
#38668=DIRECTION ( 'NONE',  ( 0.000000000000000000, 1.000000000000000000, 0.000000000000000000 ) ) ;
#38669=ADVANCED_FACE ( 'NONE', ( #53328 ), #76841, .T. ) ;
#38671=ORIENTED_EDGE ( 'NONE', *, *, #4630, .F. ) ;
#38672=CARTESIAN_POINT ( 'NONE',  ( -6.650000000000018119, 12.50000000000000000, -2.099970236277064473 ) ) ;
#38673=CARTESIAN_POINT ( 'NONE',  ( -1.850000000000033396, 2.500000000000000000, -6.248780366869526759 ) ) ;
#38674=VECTOR ( 'NONE', #81141, 1000.000000000000000 ) ;
#38675=AXIS2_PLACEMENT_3D ( 'NONE', #117500, #108987, #118178 ) ;
#38676=EDGE_CURVE ( 'NONE', #97603, #96273, #32417, .T. ) ;
#38677=DIRECTION ( 'NONE',  ( 0.000000000000000000, -0.000000000000000000, 1.000000000000000000 ) ) ;
#38678=DIRECTION ( 'NONE',  ( -0.000000000000000000, -1.000000000000000000, -0.000000000000000000 ) ) ;
#38679=EDGE_CURVE ( 'NONE', #122539, #58927, #22480, .T. ) ;
#38680=AXIS2_PLACEMENT_3D ( 'NONE', #63097, #20608, #100448 ) ;
#38681=ORIENTED_EDGE ( 'NONE', *, *, #46154, .T. ) ;
#38682=EDGE_CURVE ( 'NONE', #63649, #125318, #52662, .T. ) ;
#38683=FACE_OUTER_BOUND ( 'NONE', #104219, .T. ) ;
#38684=LINE ( 'NONE', #57661, #68567 ) ;
#38685=LINE ( 'NONE', #11114, #34621 ) ;
#38686=DIRECTION ( 'NONE',  ( 0.000000000000000000, 0.000000000000000000, -1.000000000000000000 ) ) ;
#38687=ORIENTED_EDGE ( 'NONE', *, *, #71579, .F. ) ;
#38688=CARTESIAN_POINT ( 'NONE',  ( -7.100000000000017408, 12.50000000000000000, -0.7579135962115917113 ) ) ;
#38689=ORIENTED_EDGE ( 'NONE', *, *, #34196, .T. ) ;
#38690=EDGE_CURVE ( 'NONE', #129208, #98964, #126924, .T. ) ;
#38691=DIRECTION ( 'NONE',  ( 0.000000000000000000, 0.000000000000000000, 1.000000000000000000 ) ) ;
#38692=ADVANCED_FACE ( 'NONE', ( #22591 ), #14029, .T. ) ;
#38693=VERTEX_POINT ( 'NONE', #103712 ) ;
#38694=PLANE ( 'NONE',  #128783 ) ;
#38695=CARTESIAN_POINT ( 'NONE',  ( 87.50000000000002842, -7.499999999999997335, 0.6928095518838454092 ) ) ;
#38696=EDGE_CURVE ( 'NONE', #11963, #9662, #87188, .T. ) ;
#38697=CARTESIAN_POINT ( 'NONE',  ( 7.899999999999923084, 2.500000000000000000, -0.6928203230275542523 ) ) ;
#38698=ADVANCED_FACE ( 'NONE', ( #4188 ), #64208, .T. ) ;
#38699=AXIS2_PLACEMENT_3D ( 'NONE', #69962, #70601, #50316 ) ;
#38700=CARTESIAN_POINT ( 'NONE',  ( -7.300000000000018474, 2.500000000000000000, 0.2464101615137735679 ) ) ;
#38701=ORIENTED_EDGE ( 'NONE', *, *, #8043, .T. ) ;
#38702=AXIS2_PLACEMENT_3D ( 'NONE', #118739, #9440, #70296 ) ;
#38703=DIRECTION ( 'NONE',  ( -0.000000000000000000, -1.000000000000000000, -0.000000000000000000 ) ) ;
#38704=DIRECTION ( 'NONE',  ( -0.000000000000000000, -1.000000000000000000, -0.000000000000000000 ) ) ;
#38705=CARTESIAN_POINT ( 'NONE',  ( 9.999999999999948486, 2.500000000000000000, -4.230127018922201998 ) ) ;
#38706=CIRCLE ( 'NONE', #53353, 0.06509327318403745899 ) ;
#38707=CARTESIAN_POINT ( 'NONE',  ( -6.850000000000017408, 2.500000000000000000, -1.818653347947325916 ) ) ;
#38708=CARTESIAN_POINT ( 'NONE',  ( -2.499999999999996447, 12.50000000000000000, 4.330127018922196314 ) ) ;
#38709=DIRECTION ( 'NONE',  ( 0.000000000000000000, 1.000000000000000000, 0.000000000000000000 ) ) ;
#38710=EDGE_CURVE ( 'NONE', #120555, #21815, #24498, .T. ) ;
#38711=AXIS2_PLACEMENT_3D ( 'NONE', #40830, #8267, #11980 ) ;
#38712=ORIENTED_EDGE ( 'NONE', *, *, #38627, .F. ) ;
#38713=EDGE_LOOP ( 'NONE', ( #21252, #63195, #84803, #106965 ) ) ;
#38714=AXIS2_PLACEMENT_3D ( 'NONE', #78818, #19213, #59172 ) ;
#38715=DIRECTION ( 'NONE',  ( -0.000000000000000000, -1.000000000000000000, -0.000000000000000000 ) ) ;
#38716=EDGE_LOOP ( 'NONE', ( #113800, #48859, #14993, #44222 ) ) ;
#38717=DIRECTION ( 'NONE',  ( 0.000000000000000000, -0.000000000000000000, 1.000000000000000000 ) ) ;
#38718=CONICAL_SURFACE ( 'NONE', #51222, 0.09999999999999982514, 0.003490658503988666988 ) ;
#38719=ORIENTED_EDGE ( 'NONE', *, *, #20049, .T. ) ;
#38720=VERTEX_POINT ( 'NONE', #34985 ) ;
#38721=ORIENTED_EDGE ( 'NONE', *, *, #18086, .F. ) ;
#38722=CARTESIAN_POINT ( 'NONE',  ( -3.350000000000028955, 2.500000000000000000, -2.265063509461101798 ) ) ;
#38723=AXIS2_PLACEMENT_3D ( 'NONE', #113088, #84270, #85562 ) ;
#38724=CARTESIAN_POINT ( 'NONE',  ( 7.699999999999923794, 2.500000000000000000, -3.983716857408426293 ) ) ;
#38725=CONICAL_SURFACE ( 'NONE', #78424, 0.1000000000000002554, 0.003490658503988666988 ) ;
#38726=DIRECTION ( 'NONE',  ( 0.000000000000000000, 0.000000000000000000, 1.000000000000000000 ) ) ;
#38728=FACE_OUTER_BOUND ( 'NONE', #66481, .T. ) ;
#38729=CARTESIAN_POINT ( 'NONE',  ( 14.54999999999989591, 12.50000000000000000, 2.099970236277060032 ) ) ;
#38730=CIRCLE ( 'NONE', #9453, 0.09999999999999982514 ) ;
#38731=DIRECTION ( 'NONE',  ( 0.000000000000000000, -0.000000000000000000, 1.000000000000000000 ) ) ;
#38732=CARTESIAN_POINT ( 'NONE',  ( 6.899999999999926636, 2.500000000000000000, 0.4464101615137736623 ) ) ;
#38733=DIRECTION ( 'NONE',  ( -4.274815082592931898E-19, -0.9999939076577903929, -0.003490651415223739937 ) ) ;
#38734=ORIENTED_EDGE ( 'NONE', *, *, #14093, .F. ) ;
#38735=ORIENTED_EDGE ( 'NONE', *, *, #44980, .F. ) ;
#38736=ORIENTED_EDGE ( 'NONE', *, *, #116818, .F. ) ;
#38737=DIRECTION ( 'NONE',  ( 0.000000000000000000, 0.000000000000000000, 1.000000000000000000 ) ) ;
#38738=ORIENTED_EDGE ( 'NONE', *, *, #5469, .F. ) ;
#38739=EDGE_LOOP ( 'NONE', ( #79061, #101615, #12936, #43714 ) ) ;
#38740=LINE ( 'NONE', #100211, #44105 ) ;
#38741=VECTOR ( 'NONE', #40775, 1000.000000000000000 ) ;
#38742=CARTESIAN_POINT ( 'NONE',  ( -5.450000000000019718, 2.500000000000000000, 6.495190528383297135 ) ) ;
#38743=EDGE_CURVE ( 'NONE', #23431, #30816, #48017, .T. ) ;
#38745=DIRECTION ( 'NONE',  ( 0.000000000000000000, 1.000000000000000000, 0.000000000000000000 ) ) ;
#38746=DIRECTION ( 'NONE',  ( 0.000000000000000000, 0.000000000000000000, 1.000000000000000000 ) ) ;
#38747=CARTESIAN_POINT ( 'NONE',  ( -6.900000000000019007, 2.500000000000000000, 0.3464101615137735735 ) ) ;
#38748=ORIENTED_EDGE ( 'NONE', *, *, #127322, .F. ) ;
#38749=AXIS2_PLACEMENT_3D ( 'NONE', #42051, #81959, #101618 ) ;
#38750=CARTESIAN_POINT ( 'NONE',  ( 8.549999999999924327, 12.50000000000000000, -6.841600689897077814 ) ) ;
#38751=AXIS2_PLACEMENT_3D ( 'NONE', #99202, #49469, #89379 ) ;
#38752=AXIS2_PLACEMENT_3D ( 'NONE', #28011, #69203, #109121 ) ;
#38753=ORIENTED_EDGE ( 'NONE', *, *, #38194, .T. ) ;
#38754=CARTESIAN_POINT ( 'NONE',  ( -13.54999999999999005, 2.500000000000000000, -1.918653347947324006 ) ) ;
#38755=ORIENTED_EDGE ( 'NONE', *, *, #77643, .F. ) ;
#38756=LINE ( 'NONE', #37450, #33742 ) ;
#38757=ORIENTED_EDGE ( 'NONE', *, *, #48232, .T. ) ;
#38758=EDGE_CURVE ( 'NONE', #107667, #37222, #1514, .T. ) ;
#38759=ORIENTED_EDGE ( 'NONE', *, *, #16646, .F. ) ;
#38760=DIRECTION ( 'NONE',  ( 0.000000000000000000, 0.000000000000000000, 1.000000000000000000 ) ) ;
#38761=CARTESIAN_POINT ( 'NONE',  ( 76.44220535186029508, -3.905138931494386956, -5.869652189505990769 ) ) ;
#38762=AXIS2_PLACEMENT_3D ( 'NONE', #26862, #77879, #46488 ) ;
#38763=LINE ( 'NONE', #78673, #109335 ) ;
#38764=CARTESIAN_POINT ( 'NONE',  ( -12.69999999999999218, 12.50000000000000000, 4.676537180435972552 ) ) ;
#38765=VECTOR ( 'NONE', #94188, 1000.000000000000000 ) ;
#38766=DIRECTION ( 'NONE',  ( -0.000000000000000000, -1.000000000000000000, -0.000000000000000000 ) ) ;
#38767=EDGE_LOOP ( 'NONE', ( #7276, #15895 ) ) ;
#38768=CARTESIAN_POINT ( 'NONE',  ( 6.849999999999930367, 12.50000000000000000, -6.148780366869526226 ) ) ;
#38769=CARTESIAN_POINT ( 'NONE',  ( -9.150000000000009237, 2.500000000000000000, 2.857883832488649301 ) ) ;
#38770=CARTESIAN_POINT ( 'NONE',  ( 11.04999999999991189, 2.500000000000000000, 6.048780366869521252 ) ) ;
#38771=CARTESIAN_POINT ( 'NONE',  ( -0.4000000000000401013, 2.500000000000000000, -3.637306695894650055 ) ) ;
#38772=DIRECTION ( 'NONE',  ( 0.000000000000000000, 0.000000000000000000, 1.000000000000000000 ) ) ;
#38773=ORIENTED_EDGE ( 'NONE', *, *, #90994, .F. ) ;
#38774=CIRCLE ( 'NONE', #7335, 0.06509327318403745899 ) ;
#38775=AXIS2_PLACEMENT_3D ( 'NONE', #49316, #59782, #19159 ) ;
#38776=ORIENTED_EDGE ( 'NONE', *, *, #36886, .F. ) ;
#38777=CARTESIAN_POINT ( 'NONE',  ( -6.850000000000017408, 2.500000000000000000, -6.248780366869526759 ) ) ;
#38778=EDGE_LOOP ( 'NONE', ( #80295, #122562, #66744, #47976 ) ) ;
#38779=LINE ( 'NONE', #98958, #128162 ) ;
#38780=CARTESIAN_POINT ( 'NONE',  ( -9.800000000000007816, 2.500000000000000000, -3.983716857408421852 ) ) ;
#38781=EDGE_CURVE ( 'NONE', #75194, #75250, #11982, .T. ) ;
#38782=AXIS2_PLACEMENT_3D ( 'NONE', #82963, #34520, #74431 ) ;
#38783=VERTEX_POINT ( 'NONE', #45435 ) ;
#38785=DIRECTION ( 'NONE',  ( -4.274815082592931898E-19, -0.9999939076577903929, -0.003490651415223739937 ) ) ;
#38786=CARTESIAN_POINT ( 'NONE',  ( -2.300000000000033573, 12.50000000000000000, -3.983716857408426293 ) ) ;
#38787=CIRCLE ( 'NONE', #78492, 0.06509327318403741736 ) ;
#38788=DIRECTION ( 'NONE',  ( -0.000000000000000000, -1.000000000000000000, -0.000000000000000000 ) ) ;
#38789=ORIENTED_EDGE ( 'NONE', *, *, #101453, .F. ) ;
#38790=EDGE_CURVE ( 'NONE', #70542, #116584, #74681, .T. ) ;
#38791=CIRCLE ( 'NONE', #90989, 0.06509327318403745899 ) ;
#38792=FACE_OUTER_BOUND ( 'NONE', #75030, .T. ) ;
#38793=CIRCLE ( 'NONE', #38702, 0.06509327318403745899 ) ;
#38794=EDGE_LOOP ( 'NONE', ( #59155, #9323 ) ) ;
#38795=ADVANCED_FACE ( 'NONE', ( #38187 ), #125901, .T. ) ;
#38796=EDGE_CURVE ( 'NONE', #74258, #40987, #67626, .T. ) ;
#38797=EDGE_CURVE ( 'NONE', #68062, #64597, #24598, .T. ) ;
#38798=CARTESIAN_POINT ( 'NONE',  ( 35.04033562331356677, 1.562405403454929065, -4.793261083390611077 ) ) ;
#38799=EDGE_CURVE ( 'NONE', #74146, #79205, #127222, .T. ) ;
#38800=FACE_OUTER_BOUND ( 'NONE', #49086, .T. ) ;
#38801=DIRECTION ( 'NONE',  ( 0.000000000000000000, 0.000000000000000000, -1.000000000000000000 ) ) ;
#38802=VECTOR ( 'NONE', #3457, 1000.000000000000000 ) ;
#38803=CONICAL_SURFACE ( 'NONE', #7361, 0.1000000000000002554, 0.003490658503988666988 ) ;
#38804=EDGE_LOOP ( 'NONE', ( #87377, #84539, #1014, #124118 ) ) ;
#38805=VECTOR ( 'NONE', #93778, 1000.000000000000000 ) ;
#38806=CARTESIAN_POINT ( 'NONE',  ( -6.450000000000019718, 12.50000000000000000, -6.148780366869526226 ) ) ;
#38807=CIRCLE ( 'NONE', #76433, 0.1000000000000000472 ) ;
#38808=VERTEX_POINT ( 'NONE', #76825 ) ;
#38809=DIRECTION ( 'NONE',  ( 0.000000000000000000, 0.000000000000000000, 1.000000000000000000 ) ) ;
#38810=DIRECTION ( 'NONE',  ( 0.000000000000000000, 0.000000000000000000, 1.000000000000000000 ) ) ;
#38811=EDGE_CURVE ( 'NONE', #21177, #112816, #39304, .T. ) ;
#38812=CARTESIAN_POINT ( 'NONE',  ( 0.5999999999999621192, 12.50000000000000000, 0.2813168883297384459 ) ) ;
#38813=ORIENTED_EDGE ( 'NONE', *, *, #111519, .F. ) ;
#38814=EDGE_CURVE ( 'NONE', #119487, #74873, #51801, .T. ) ;
#38815=CIRCLE ( 'NONE', #107736, 0.09999999999999982514 ) ;
#38816=AXIS2_PLACEMENT_3D ( 'NONE', #93093, #63627, #51875 ) ;
#38817=CARTESIAN_POINT ( 'NONE',  ( -5.650000000000019895, 12.50000000000000000, 6.083687093685482772 ) ) ;
#38818=EDGE_CURVE ( 'NONE', #83051, #83715, #77459, .T. ) ;
#38819=AXIS2_PLACEMENT_3D ( 'NONE', #93752, #23078, #5356 ) ;
#38820=DIRECTION ( 'NONE',  ( 0.000000000000000000, 0.000000000000000000, -1.000000000000000000 ) ) ;
#38821=ORIENTED_EDGE ( 'NONE', *, *, #124057, .T. ) ;
#38822=CARTESIAN_POINT ( 'NONE',  ( 9.149999999999916866, 2.500000000000000000, -2.857883832488653741 ) ) ;
#38823=VERTEX_POINT ( 'NONE', #7417 ) ;
#38824=CARTESIAN_POINT ( 'NONE',  ( 8.099999999999923261, 12.50000000000000000, 3.983716857408420076 ) ) ;
#38825=EDGE_LOOP ( 'NONE', ( #74035, #115540, #92055, #14706 ) ) ;
#38826=DIRECTION ( 'NONE',  ( -0.000000000000000000, -1.000000000000000000, -0.000000000000000000 ) ) ;
#38827=DIRECTION ( 'NONE',  ( 0.000000000000000000, 1.000000000000000000, 0.000000000000000000 ) ) ;
#38828=ORIENTED_EDGE ( 'NONE', *, *, #4158, .T. ) ;
#38829=VERTEX_POINT ( 'NONE', #117347 ) ;
#38830=DIRECTION ( 'NONE',  ( 0.000000000000000000, 0.000000000000000000, -1.000000000000000000 ) ) ;
#38831=CARTESIAN_POINT ( 'NONE',  ( 0.6499999999999543920, 12.50000000000000000, 6.776507416713035248 ) ) ;
#38832=CONICAL_SURFACE ( 'NONE', #57594, 0.09999999999999982514, 0.003490658503988666988 ) ;
#38833=EDGE_LOOP ( 'NONE', ( #46889, #63289 ) ) ;
#38834=DIRECTION ( 'NONE',  ( 0.000000000000000000, 0.000000000000000000, -1.000000000000000000 ) ) ;
#38835=PLANE ( 'NONE',  #118251 ) ;
#38836=CARTESIAN_POINT ( 'NONE',  ( 10.84999999999990905, 2.500000000000000000, 2.165063509461097713 ) ) ;
#38838=CARTESIAN_POINT ( 'NONE',  ( -2.700000000000029932, 12.50000000000000000, -0.3464101615137782364 ) ) ;
#38840=AXIS2_PLACEMENT_3D ( 'NONE', #20317, #49792, #60263 ) ;
#38841=FACE_OUTER_BOUND ( 'NONE', #89490, .T. ) ;
#38842=AXIS2_PLACEMENT_3D ( 'NONE', #116731, #44796, #14655 ) ;
#38843=AXIS2_PLACEMENT_3D ( 'NONE', #31878, #113006, #23325 ) ;
#38844=ORIENTED_EDGE ( 'NONE', *, *, #32499, .T. ) ;
#38845=ORIENTED_EDGE ( 'NONE', *, *, #69788, .F. ) ;
#38846=ORIENTED_EDGE ( 'NONE', *, *, #3910, .F. ) ;
#38847=ORIENTED_EDGE ( 'NONE', *, *, #74665, .T. ) ;
#38848=CARTESIAN_POINT ( 'NONE',  ( -2.900000000000030109, 2.500000000000000000, 0.6928203230275494784 ) ) ;
#38849=CARTESIAN_POINT ( 'NONE',  ( -10.60000000000000142, 12.50000000000000000, 3.983716857408420964 ) ) ;
#38850=DIRECTION ( 'NONE',  ( 0.000000000000000000, 0.000000000000000000, -1.000000000000000000 ) ) ;
#38851=EDGE_LOOP ( 'NONE', ( #74664, #27304 ) ) ;
#38852=FACE_BOUND ( 'NONE', #126150, .T. ) ;
#38853=ORIENTED_EDGE ( 'NONE', *, *, #59792, .F. ) ;
#38854=EDGE_CURVE ( 'NONE', #75500, #86861, #85348, .T. ) ;
#38855=CARTESIAN_POINT ( 'NONE',  ( -5.650000000000019895, 12.50000000000000000, 6.841600689897072485 ) ) ;
#38857=AXIS2_PLACEMENT_3D ( 'NONE', #62781, #103349, #51674 ) ;
#38858=ADVANCED_FACE ( 'NONE', ( #57172 ), #5795, .T. ) ;
#38859=DIRECTION ( 'NONE',  ( 0.000000000000000000, 0.000000000000000000, 1.000000000000000000 ) ) ;
#38860=DIRECTION ( 'NONE',  ( 0.000000000000000000, -0.9999939076577903929, 0.003490651415223739937 ) ) ;
#38861=AXIS2_PLACEMENT_3D ( 'NONE', #52182, #92759, #69892 ) ;
#38862=EDGE_CURVE ( 'NONE', #28471, #86078, #26747, .T. ) ;
#38863=CARTESIAN_POINT ( 'NONE',  ( 2.299999999999948752, 12.50000000000000000, 0.3464101615137735735 ) ) ;
#38864=DIRECTION ( 'NONE',  ( 0.000000000000000000, 0.000000000000000000, 1.000000000000000000 ) ) ;
#38865=CARTESIAN_POINT ( 'NONE',  ( -8.749999999999975131, 2.500000000000000000, -2.265063509461101798 ) ) ;
#38866=CARTESIAN_POINT ( 'NONE',  ( -9.600000000000006750, 12.50000000000000000, 5.022947341949748790 ) ) ;
#38867=FACE_OUTER_BOUND ( 'NONE', #23849, .T. ) ;
#38868=CARTESIAN_POINT ( 'NONE',  ( -10.40000000000000213, 2.500000000000000000, -2.276824562219559311E-15 ) ) ;
#38869=EDGE_CURVE ( 'NONE', #63695, #98092, #64306, .T. ) ;
#38870=AXIS2_PLACEMENT_3D ( 'NONE', #23171, #12066, #12694 ) ;
#38871=ORIENTED_EDGE ( 'NONE', *, *, #108437, .T. ) ;
#38872=VERTEX_POINT ( 'NONE', #105642 ) ;
#38873=VECTOR ( 'NONE', #63629, 1000.000000000000000 ) ;
#38874=ORIENTED_EDGE ( 'NONE', *, *, #77695, .T. ) ;
#38875=ORIENTED_EDGE ( 'NONE', *, *, #1946, .T. ) ;
#38876=FACE_OUTER_BOUND ( 'NONE', #126713, .T. ) ;
#38877=CARTESIAN_POINT ( 'NONE',  ( -16.50000000000000000, 1.500000000000000000, 1.734723475976807094E-15 ) ) ;
#38878=ORIENTED_EDGE ( 'NONE', *, *, #128717, .T. ) ;
#38879=ORIENTED_EDGE ( 'NONE', *, *, #52274, .F. ) ;
#38880=EDGE_LOOP ( 'NONE', ( #52776, #21406 ) ) ;
#38881=ADVANCED_FACE ( 'NONE', ( #17889 ), #6752, .T. ) ;
#38882=DIRECTION ( 'NONE',  ( -0.000000000000000000, 1.000000000000000000, -0.000000000000000000 ) ) ;
#38883=DIRECTION ( 'NONE',  ( 0.000000000000000000, 1.000000000000000000, 0.000000000000000000 ) ) ;
#38884=DIRECTION ( 'NONE',  ( 0.000000000000000000, 0.000000000000000000, -1.000000000000000000 ) ) ;
#38885=LINE ( 'NONE', #127242, #31242 ) ;
#38886=CARTESIAN_POINT ( 'NONE',  ( 3.549999999999941203, 2.500000000000000000, 6.148780366869520897 ) ) ;
#38887=DIRECTION ( 'NONE',  ( -0.000000000000000000, 1.000000000000000000, -0.000000000000000000 ) ) ;
#38889=ADVANCED_FACE ( 'NONE', ( #65040 ), #53852, .T. ) ;
#38890=ORIENTED_EDGE ( 'NONE', *, *, #86315, .T. ) ;
#38891=FACE_OUTER_BOUND ( 'NONE', #11544, .T. ) ;
#38892=VERTEX_POINT ( 'NONE', #25778 ) ;
#38893=AXIS2_PLACEMENT_3D ( 'NONE', #126569, #118024, #36905 ) ;
#38895=ORIENTED_EDGE ( 'NONE', *, *, #44711, .T. ) ;
#38896=CONICAL_SURFACE ( 'NONE', #7451, 0.1000000000000002554, 0.003490658503988666988 ) ;
#38897=DIRECTION ( 'NONE',  ( -0.000000000000000000, 1.000000000000000000, -0.000000000000000000 ) ) ;
#38898=ORIENTED_EDGE ( 'NONE', *, *, #117678, .F. ) ;
#38899=EDGE_LOOP ( 'NONE', ( #100620, #2973 ) ) ;
#38900=DIRECTION ( 'NONE',  ( -0.000000000000000000, -1.000000000000000000, -0.000000000000000000 ) ) ;
#38901=DIRECTION ( 'NONE',  ( 0.000000000000000000, 1.000000000000000000, 0.000000000000000000 ) ) ;
#38902=DIRECTION ( 'NONE',  ( 0.000000000000000000, 1.000000000000000000, 0.000000000000000000 ) ) ;
#38903=EDGE_CURVE ( 'NONE', #102323, #33917, #15942, .T. ) ;
#38904=CARTESIAN_POINT ( 'NONE',  ( 11.64999999999990798, 2.500000000000000000, 7.188010851410848723 ) ) ;
#38905=LINE ( 'NONE', #61591, #108278 ) ;
#38906=ORIENTED_EDGE ( 'NONE', *, *, #98847, .T. ) ;
#38907=DIRECTION ( 'NONE',  ( 0.000000000000000000, 0.000000000000000000, 1.000000000000000000 ) ) ;
#38908=CIRCLE ( 'NONE', #118284, 0.1000000000000002554 ) ;
#38909=AXIS2_PLACEMENT_3D ( 'NONE', #84546, #75358, #95655 ) ;
#38910=EDGE_LOOP ( 'NONE', ( #73720, #58796, #122240, #123581 ) ) ;
#38911=CARTESIAN_POINT ( 'NONE',  ( -3.550000000000027356, 12.50000000000000000, 1.883746621131358934 ) ) ;
#38912=CIRCLE ( 'NONE', #57761, 0.1000000000000000472 ) ;
#38913=EDGE_LOOP ( 'NONE', ( #80861, #60261, #59649, #5505 ) ) ;
#38915=DIRECTION ( 'NONE',  ( 0.000000000000000000, 0.000000000000000000, 1.000000000000000000 ) ) ;
#38916=AXIS2_PLACEMENT_3D ( 'NONE', #115036, #95417, #84942 ) ;
#38917=ORIENTED_EDGE ( 'NONE', *, *, #126681, .F. ) ;
#38918=DIRECTION ( 'NONE',  ( 0.000000000000000000, 1.000000000000000000, 0.000000000000000000 ) ) ;
#38919=EDGE_CURVE ( 'NONE', #54886, #54702, #89444, .T. ) ;
#38921=VERTEX_POINT ( 'NONE', #120612 ) ;
#38922=CARTESIAN_POINT ( 'NONE',  ( 5.649999999999934630, 12.50000000000000000, 6.148780366869520897 ) ) ;
#38923=ORIENTED_EDGE ( 'NONE', *, *, #46268, .F. ) ;
#38924=ADVANCED_FACE ( 'NONE', ( #11292 ), #124948, .T. ) ;
#38925=ORIENTED_EDGE ( 'NONE', *, *, #61544, .T. ) ;
#38926=DIRECTION ( 'NONE',  ( 1.000000000000000000, 0.000000000000000000, 0.000000000000000000 ) ) ;
#38927=DIRECTION ( 'NONE',  ( -0.000000000000000000, -1.000000000000000000, -0.000000000000000000 ) ) ;
#38928=CARTESIAN_POINT ( 'NONE',  ( 5.399999999999934630, 2.500000000000000000, 0.5928203230275495006 ) ) ;
#38929=AXIS2_PLACEMENT_3D ( 'NONE', #42549, #111914, #92257 ) ;
#38930=CARTESIAN_POINT ( 'NONE',  ( 1.849999999999949019, 2.500000000000000000, 6.841600689897072485 ) ) ;
#38934=AXIS2_PLACEMENT_3D ( 'NONE', #64741, #123032, #104655 ) ;
#38935=AXIS2_PLACEMENT_3D ( 'NONE', #42700, #93073, #123785 ) ;
#38936=ORIENTED_EDGE ( 'NONE', *, *, #7723, .F. ) ;
#38937=CONICAL_SURFACE ( 'NONE', #3391, 0.1000000000000000472, 0.003490658503988666988 ) ;
#38938=DIRECTION ( 'NONE',  ( -0.000000000000000000, -1.000000000000000000, -0.000000000000000000 ) ) ;
#38939=DIRECTION ( 'NONE',  ( -0.000000000000000000, -1.000000000000000000, -0.000000000000000000 ) ) ;
#38940=VECTOR ( 'NONE', #72616, 1000.000000000000000 ) ;
#38941=EDGE_CURVE ( 'NONE', #25583, #118034, #110147, .T. ) ;
#38942=ORIENTED_EDGE ( 'NONE', *, *, #73817, .T. ) ;
#38943=DIRECTION ( 'NONE',  ( -0.000000000000000000, 1.000000000000000000, -0.000000000000000000 ) ) ;
#38944=DIRECTION ( 'NONE',  ( -4.274815082592931898E-19, -0.9999939076577903929, -0.003490651415223739937 ) ) ;
#38945=CARTESIAN_POINT ( 'NONE',  ( 3.749999999999940492, 2.500000000000000000, 5.902370205355745192 ) ) ;
#38946=DIRECTION ( 'NONE',  ( 0.000000000000000000, 1.000000000000000000, 0.000000000000000000 ) ) ;
#38947=DIRECTION ( 'NONE',  ( 0.000000000000000000, 0.000000000000000000, 1.000000000000000000 ) ) ;
#38948=VERTEX_POINT ( 'NONE', #100333 ) ;
#38949=AXIS2_PLACEMENT_3D ( 'NONE', #52305, #2538, #111203 ) ;
#38950=EDGE_CURVE ( 'NONE', #11046, #102186, #47597, .T. ) ;
#38951=LINE ( 'NONE', #78862, #2004 ) ;
#38952=CIRCLE ( 'NONE', #70226, 0.1000000000000000472 ) ;
#38953=DIRECTION ( 'NONE',  ( 0.000000000000000000, 0.000000000000000000, 1.000000000000000000 ) ) ;
#38954=DIRECTION ( 'NONE',  ( 0.000000000000000000, 1.000000000000000000, 0.000000000000000000 ) ) ;
#38955=EDGE_CURVE ( 'NONE', #128693, #66202, #68506, .T. ) ;
#38956=ADVANCED_FACE ( 'NONE', ( #79410 ), #30961, .T. ) ;
#38957=EDGE_CURVE ( 'NONE', #82926, #3365, #28815, .T. ) ;
#38958=EDGE_CURVE ( 'NONE', #87862, #83631, #60222, .T. ) ;
#38959=ORIENTED_EDGE ( 'NONE', *, *, #7139, .F. ) ;
#38960=PLANE ( 'NONE',  #17606 ) ;
#38961=VERTEX_POINT ( 'NONE', #69568 ) ;
#38962=VERTEX_POINT ( 'NONE', #18538 ) ;
#38963=DIRECTION ( 'NONE',  ( -0.000000000000000000, -1.000000000000000000, -0.000000000000000000 ) ) ;
#38964=EDGE_CURVE ( 'NONE', #101462, #35406, #89852, .T. ) ;
#38965=ADVANCED_FACE ( 'NONE', ( #59122 ), #91499, .T. ) ;
#38966=ORIENTED_EDGE ( 'NONE', *, *, #39800, .F. ) ;
#38967=DIRECTION ( 'NONE',  ( 0.000000000000000000, 1.000000000000000000, 0.000000000000000000 ) ) ;
#38968=FACE_OUTER_BOUND ( 'NONE', #11138, .T. ) ;
#38969=EDGE_CURVE ( 'NONE', #102800, #17230, #78114, .T. ) ;
#38970=VERTEX_POINT ( 'NONE', #59786 ) ;
#38971=ADVANCED_FACE ( 'NONE', ( #833 ), #80700, .T. ) ;
#38972=DIRECTION ( 'NONE',  ( 0.000000000000000000, 0.000000000000000000, 1.000000000000000000 ) ) ;
#38973=ADVANCED_FACE ( 'NONE', ( #49319 ), #55976, .T. ) ;
#38974=DIRECTION ( 'NONE',  ( 0.000000000000000000, 0.000000000000000000, 1.000000000000000000 ) ) ;
#38975=ORIENTED_EDGE ( 'NONE', *, *, #49029, .F. ) ;
#38977=DIRECTION ( 'NONE',  ( 0.000000000000000000, 0.000000000000000000, 1.000000000000000000 ) ) ;
#38978=ADVANCED_FACE ( 'NONE', ( #28373 ), #129190, .T. ) ;
#38979=VERTEX_POINT ( 'NONE', #78773 ) ;
#38980=VECTOR ( 'NONE', #112090, 1000.000000000000000 ) ;
#38981=ORIENTED_EDGE ( 'NONE', *, *, #10316, .F. ) ;
#38982=CIRCLE ( 'NONE', #120427, 0.06509327318403745899 ) ;
#38983=ORIENTED_EDGE ( 'NONE', *, *, #59551, .T. ) ;
#38984=LINE ( 'NONE', #69038, #33707 ) ;
#38985=DIRECTION ( 'NONE',  ( 0.000000000000000000, 0.000000000000000000, 1.000000000000000000 ) ) ;
#38986=CARTESIAN_POINT ( 'NONE',  ( 0.1999999999999571565, 12.50000000000000000, 3.983716857408420076 ) ) ;
#38987=FACE_BOUND ( 'NONE', #29458, .T. ) ;
#38988=ORIENTED_EDGE ( 'NONE', *, *, #10516, .T. ) ;
#38989=FACE_OUTER_BOUND ( 'NONE', #24062, .T. ) ;
#38990=DIRECTION ( 'NONE',  ( -0.000000000000000000, 1.000000000000000000, -0.000000000000000000 ) ) ;
#38991=ORIENTED_EDGE ( 'NONE', *, *, #122452, .T. ) ;
#38992=CIRCLE ( 'NONE', #47285, 0.09999999999999982514 ) ;
#38993=CARTESIAN_POINT ( 'NONE',  ( -11.64999999999999858, 2.500000000000000000, -1.572243186433546214 ) ) ;
#38995=DIRECTION ( 'NONE',  ( 0.000000000000000000, 0.000000000000000000, 1.000000000000000000 ) ) ;
#38996=CARTESIAN_POINT ( 'NONE',  ( -10.65000000000000213, 12.50000000000000000, 1.753560074763284016 ) ) ;
#38997=DIRECTION ( 'NONE',  ( 0.000000000000000000, 0.000000000000000000, 1.000000000000000000 ) ) ;
#38998=PLANE ( 'NONE',  #116076 ) ;
#38999=DIRECTION ( 'NONE',  ( 0.000000000000000000, 0.000000000000000000, -1.000000000000000000 ) ) ;
#39000=AXIS2_PLACEMENT_3D ( 'NONE', #23774, #63698, #34250 ) ;
#39001=VECTOR ( 'NONE', #64768, 1000.000000000000000 ) ;
#39002=EDGE_LOOP ( 'NONE', ( #75294, #30840 ) ) ;
#39003=ORIENTED_EDGE ( 'NONE', *, *, #45302, .F. ) ;
#39004=VERTEX_POINT ( 'NONE', #118667 ) ;
#39005=EDGE_LOOP ( 'NONE', ( #75942, #35704, #129331, #10435 ) ) ;
#39006=EDGE_LOOP ( 'NONE', ( #69383, #98482, #121285, #77705 ) ) ;
#39007=DIRECTION ( 'NONE',  ( 0.000000000000000000, 0.000000000000000000, -1.000000000000000000 ) ) ;
#39008=FACE_OUTER_BOUND ( 'NONE', #33451, .T. ) ;
#39009=EDGE_LOOP ( 'NONE', ( #93156, #127207, #121217, #88054 ) ) ;
#39010=FACE_BOUND ( 'NONE', #27301, .T. ) ;
#39011=DIRECTION ( 'NONE',  ( 0.000000000000000000, 1.000000000000000000, 0.000000000000000000 ) ) ;
#39013=CARTESIAN_POINT ( 'NONE',  ( -4.550000000000022915, 2.500000000000000000, 2.065063509461097624 ) ) ;
#39014=EDGE_CURVE ( 'NONE', #71566, #108669, #58064, .T. ) ;
#39015=DIRECTION ( 'NONE',  ( 0.000000000000000000, 0.000000000000000000, 1.000000000000000000 ) ) ;
#39016=CARTESIAN_POINT ( 'NONE',  ( -15.59999999999998010, 2.500000000000000000, 0.2464101615137759549 ) ) ;
#39017=DIRECTION ( 'NONE',  ( 0.000000000000000000, 1.000000000000000000, 0.000000000000000000 ) ) ;
#39018=AXIS2_PLACEMENT_3D ( 'NONE', #120296, #98695, #30637 ) ;
#39019=ORIENTED_EDGE ( 'NONE', *, *, #108512, .F. ) ;
#39020=EDGE_CURVE ( 'NONE', #94819, #69257, #114475, .T. ) ;
#39021=VERTEX_POINT ( 'NONE', #102888 ) ;
#39022=VECTOR ( 'NONE', #48769, 1000.000000000000000 ) ;
#39023=ORIENTED_EDGE ( 'NONE', *, *, #114548, .T. ) ;
#39024=ORIENTED_EDGE ( 'NONE', *, *, #129566, .T. ) ;
#39025=CARTESIAN_POINT ( 'NONE',  ( 8.549999999999918998, 2.500000000000000000, -1.918653347947326004 ) ) ;
#39026=CARTESIAN_POINT ( 'NONE',  ( -5.650000000000023448, 12.50000000000000000, -6.083687093685488989 ) ) ;
#39027=CARTESIAN_POINT ( 'NONE',  ( 10.84999999999991260, 2.500000000000000000, 7.188010851410848723 ) ) ;
#39028=ORIENTED_EDGE ( 'NONE', *, *, #123164, .F. ) ;
#39029=CARTESIAN_POINT ( 'NONE',  ( 4.149999999999939959, 12.50000000000000000, 1.407149913249508000 ) ) ;
#39030=CONICAL_SURFACE ( 'NONE', #61989, 0.09999999999999982514, 0.003490658503988666988 ) ;
#39031=VECTOR ( 'NONE', #32233, 1000.000000000000000 ) ;
#39032=CARTESIAN_POINT ( 'NONE',  ( -7.300000000000016698, 2.500000000000000000, -4.576537180435978236 ) ) ;
#39033=AXIS2_PLACEMENT_3D ( 'NONE', #3863, #83087, #94177 ) ;
#39034=DIRECTION ( 'NONE',  ( 0.000000000000000000, 0.000000000000000000, 1.000000000000000000 ) ) ;
#39036=LINE ( 'NONE', #38377, #4838 ) ;
#39037=CARTESIAN_POINT ( 'NONE',  ( 1.249999999999988454, 2.500000000000000000, -2.265063509461101798 ) ) ;
#39038=CARTESIAN_POINT ( 'NONE',  ( 9.349999999999919709, 12.50000000000000000, -6.841600689897078702 ) ) ;
#39039=VERTEX_POINT ( 'NONE', #102267 ) ;
#39040=DIRECTION ( 'NONE',  ( 0.000000000000000000, 0.000000000000000000, 1.000000000000000000 ) ) ;
#39041=AXIS2_PLACEMENT_3D ( 'NONE', #68884, #106241, #16546 ) ;
#39042=ORIENTED_EDGE ( 'NONE', *, *, #123411, .T. ) ;
#39043=AXIS2_PLACEMENT_3D ( 'NONE', #15794, #55091, #55728 ) ;
#39044=ORIENTED_EDGE ( 'NONE', *, *, #127638, .F. ) ;
#39045=DIRECTION ( 'NONE',  ( 0.000000000000000000, 1.000000000000000000, 0.000000000000000000 ) ) ;
#39046=DIRECTION ( 'NONE',  ( 0.000000000000000000, 0.000000000000000000, 1.000000000000000000 ) ) ;
#39047=DIRECTION ( 'NONE',  ( -4.274815082592931898E-19, -0.9999939076577903929, -0.003490651415223739937 ) ) ;
#39048=ORIENTED_EDGE ( 'NONE', *, *, #107208, .T. ) ;
#39049=ORIENTED_EDGE ( 'NONE', *, *, #5381, .F. ) ;
#39050=EDGE_CURVE ( 'NONE', #46879, #109098, #37225, .T. ) ;
#39051=FACE_OUTER_BOUND ( 'NONE', #86164, .T. ) ;
#39052=DIRECTION ( 'NONE',  ( 0.000000000000000000, 0.000000000000000000, -1.000000000000000000 ) ) ;
#39053=DIRECTION ( 'NONE',  ( 0.000000000000000000, 0.000000000000000000, -1.000000000000000000 ) ) ;
#39054=ORIENTED_EDGE ( 'NONE', *, *, #35571, .F. ) ;
#39055=DIRECTION ( 'NONE',  ( 0.000000000000000000, 1.000000000000000000, 0.000000000000000000 ) ) ;
#39057=DIRECTION ( 'NONE',  ( 0.000000000000000000, 0.000000000000000000, -1.000000000000000000 ) ) ;
#39058=ORIENTED_EDGE ( 'NONE', *, *, #11476, .T. ) ;
#39059=DIRECTION ( 'NONE',  ( 0.000000000000000000, 0.000000000000000000, -1.000000000000000000 ) ) ;
#39060=FACE_OUTER_BOUND ( 'NONE', #71018, .T. ) ;
#39061=DIRECTION ( 'NONE',  ( 0.000000000000000000, 0.000000000000000000, 1.000000000000000000 ) ) ;
#39062=ADVANCED_FACE ( 'NONE', ( #31592 ), #70569, .T. ) ;
#39063=EDGE_CURVE ( 'NONE', #37898, #86156, #30882, .T. ) ;
#39064=FACE_OUTER_BOUND ( 'NONE', #33690, .T. ) ;
#39065=ORIENTED_EDGE ( 'NONE', *, *, #70663, .T. ) ;
#39066=CARTESIAN_POINT ( 'NONE',  ( -9.150000000000005684, 12.50000000000000000, 6.495190528383297135 ) ) ;
#39067=AXIS2_PLACEMENT_3D ( 'NONE', #51730, #81187, #35 ) ;
#39068=AXIS2_PLACEMENT_3D ( 'NONE', #37310, #126970, #27453 ) ;
#39069=ORIENTED_EDGE ( 'NONE', *, *, #26593, .F. ) ;
#39070=ORIENTED_EDGE ( 'NONE', *, *, #113997, .F. ) ;
#39071=ADVANCED_FACE ( 'NONE', ( #51881 ), #45354, .T. ) ;
#39072=FACE_OUTER_BOUND ( 'NONE', #76505, .T. ) ;
#39073=CARTESIAN_POINT ( 'NONE',  ( 3.749999999999942268, 2.500000000000000000, -1.472243186433550122 ) ) ;
#39074=CARTESIAN_POINT ( 'NONE',  ( -6.900000000000019007, 2.500000000000000000, -4.576537180435978236 ) ) ;
#39075=DIRECTION ( 'NONE',  ( 0.000000000000000000, 0.000000000000000000, -1.000000000000000000 ) ) ;
#39076=CARTESIAN_POINT ( 'NONE',  ( 3.349999999999943689, 12.50000000000000000, 2.165063509461097713 ) ) ;
#39077=FACE_OUTER_BOUND ( 'NONE', #13167, .T. ) ;
#39078=CONICAL_SURFACE ( 'NONE', #51581, 0.1000000000000002554, 0.003490658503988666988 ) ;
#39079=DIRECTION ( 'NONE',  ( 0.000000000000000000, 0.000000000000000000, 1.000000000000000000 ) ) ;
#39080=FACE_OUTER_BOUND ( 'NONE', #51825, .T. ) ;
#39081=PLANE ( 'NONE',  #46343 ) ;
#39082=AXIS2_PLACEMENT_3D ( 'NONE', #19015, #28866, #86477 ) ;
#39083=CONICAL_SURFACE ( 'NONE', #112222, 0.1000000000000002554, 0.003490658503988666988 ) ;
#39084=AXIS2_PLACEMENT_3D ( 'NONE', #126558, #27689, #77447 ) ;
#39085=ORIENTED_EDGE ( 'NONE', *, *, #83136, .F. ) ;
#39086=CARTESIAN_POINT ( 'NONE',  ( -2.900000000000030109, 12.50000000000000000, 0.6928203230275494784 ) ) ;
#39087=CARTESIAN_POINT ( 'NONE',  ( 8.749999999999957367, 12.50000000000000000, -6.430097255199264339 ) ) ;
#39088=CARTESIAN_POINT ( 'NONE',  ( 11.44999999999990692, 2.500000000000000000, -6.741600689897078169 ) ) ;
#39089=FACE_OUTER_BOUND ( 'NONE', #107756, .T. ) ;
#39090=DIRECTION ( 'NONE',  ( -0.000000000000000000, -1.000000000000000000, -0.000000000000000000 ) ) ;
#39091=VERTEX_POINT ( 'NONE', #81340 ) ;
#39092=CARTESIAN_POINT ( 'NONE',  ( -3.950000000000024603, 12.50000000000000000, -2.511473670974877948 ) ) ;
#39093=EDGE_CURVE ( 'NONE', #120916, #95574, #11871, .T. ) ;
#39094=DIRECTION ( 'NONE',  ( 0.000000000000000000, 0.000000000000000000, 1.000000000000000000 ) ) ;
#39095=DIRECTION ( 'NONE',  ( 0.000000000000000000, 0.000000000000000000, -1.000000000000000000 ) ) ;
#39096=EDGE_LOOP ( 'NONE', ( #47477, #96853 ) ) ;
#39097=EDGE_CURVE ( 'NONE', #82797, #54150, #93097, .T. ) ;
#39098=AXIS2_PLACEMENT_3D ( 'NONE', #40300, #67134, #39034 ) ;
#39100=ADVANCED_FACE ( 'NONE', ( #11937 ), #118482, .T. ) ;
#39101=EDGE_LOOP ( 'NONE', ( #86976, #106788, #94077, #96714 ) ) ;
#39102=VECTOR ( 'NONE', #57009, 1000.000000000000000 ) ;
#39103=DIRECTION ( 'NONE',  ( 0.000000000000000000, -0.000000000000000000, 1.000000000000000000 ) ) ;
#39104=AXIS2_PLACEMENT_3D ( 'NONE', #16540, #46040, #74201 ) ;
#39105=ORIENTED_EDGE ( 'NONE', *, *, #58717, .F. ) ;
#39106=ORIENTED_EDGE ( 'NONE', *, *, #5483, .T. ) ;
#39107=VERTEX_POINT ( 'NONE', #14502 ) ;
#39108=DIRECTION ( 'NONE',  ( 0.000000000000000000, 0.000000000000000000, 1.000000000000000000 ) ) ;
#39109=EDGE_CURVE ( 'NONE', #114232, #33730, #125034, .T. ) ;
#39110=ADVANCED_FACE ( 'NONE', ( #91796 ), #2109, .T. ) ;
#39111=EDGE_CURVE ( 'NONE', #120522, #54801, #56073, .T. ) ;
#39112=AXIS2_PLACEMENT_3D ( 'NONE', #57986, #26587, #65854 ) ;
#39113=CARTESIAN_POINT ( 'NONE',  ( -4.200000000000025935, 2.500000000000000000, -0.1000000000000023925 ) ) ;
#39114=PLANE ( 'NONE',  #117290 ) ;
#39115=AXIS2_PLACEMENT_3D ( 'NONE', #27360, #57492, #74064 ) ;
#39116=DIRECTION ( 'NONE',  ( 0.000000000000000000, 0.000000000000000000, 1.000000000000000000 ) ) ;
#39117=ORIENTED_EDGE ( 'NONE', *, *, #73935, .T. ) ;
#39118=CIRCLE ( 'NONE', #5615, 0.06509327318403745899 ) ;
#39119=ADVANCED_FACE ( 'NONE', ( #121256 ), #71503, .T. ) ;
#39120=DIRECTION ( 'NONE',  ( 0.000000000000000000, 0.000000000000000000, 1.000000000000000000 ) ) ;
#39121=EDGE_LOOP ( 'NONE', ( #7748, #110547 ) ) ;
#39122=CARTESIAN_POINT ( 'NONE',  ( -6.450000000000014388, 12.50000000000000000, 6.148780366869520897 ) ) ;
#39123=CARTESIAN_POINT ( 'NONE',  ( 18.87984495337378732, -0.5408627091910553908, -4.542689527610523470 ) ) ;
#39124=CARTESIAN_POINT ( 'NONE',  ( -1.650000000000034772, 2.500000000000000000, 2.265063509461097357 ) ) ;
#39125=FACE_OUTER_BOUND ( 'NONE', #1083, .T. ) ;
#39126=AXIS2_PLACEMENT_3D ( 'NONE', #96150, #26774, #66046 ) ;
#39127=CARTESIAN_POINT ( 'NONE',  ( 5.399999999999934630, 12.50000000000000000, 0.6277270498435120194 ) ) ;
#39128=EDGE_CURVE ( 'NONE', #114933, #98804, #87368, .T. ) ;
#39129=AXIS2_PLACEMENT_3D ( 'NONE', #119929, #79369, #29607 ) ;
#39130=ORIENTED_EDGE ( 'NONE', *, *, #127740, .F. ) ;
#39131=CIRCLE ( 'NONE', #18159, 0.1000000000000000472 ) ;
#39132=CIRCLE ( 'NONE', #20234, 0.06509327318403745899 ) ;
#39133=EDGE_LOOP ( 'NONE', ( #22837, #71185, #109986, #8557 ) ) ;
#39134=ORIENTED_EDGE ( 'NONE', *, *, #47537, .F. ) ;
#39135=VERTEX_POINT ( 'NONE', #103560 ) ;
#39136=ORIENTED_EDGE ( 'NONE', *, *, #108084, .F. ) ;
#39137=DIRECTION ( 'NONE',  ( 0.000000000000000000, -0.9999939076577903929, 0.003490651415223739937 ) ) ;
#39138=DIRECTION ( 'NONE',  ( -4.274815082592931898E-19, -0.9999939076577903929, -0.003490651415223739937 ) ) ;
#39139=FACE_OUTER_BOUND ( 'NONE', #15164, .T. ) ;
#39140=FACE_BOUND ( 'NONE', #110795, .T. ) ;
#39141=CARTESIAN_POINT ( 'NONE',  ( 8.949999999999921130, 2.500000000000000000, -6.941600689897078347 ) ) ;
#39143=FACE_OUTER_BOUND ( 'NONE', #45136, .T. ) ;
#39144=DIRECTION ( 'NONE',  ( 0.000000000000000000, 1.000000000000000000, 0.000000000000000000 ) ) ;
#39145=DIRECTION ( 'NONE',  ( -0.000000000000000000, 1.000000000000000000, -0.000000000000000000 ) ) ;
#39146=CARTESIAN_POINT ( 'NONE',  ( 6.249999999999967137, 12.50000000000000000, 6.495190528383297135 ) ) ;
#39147=VECTOR ( 'NONE', #126747, 1000.000000000000000 ) ;
#39148=CARTESIAN_POINT ( 'NONE',  ( 11.24999999999994493, 2.500000000000000000, 6.495190528383297135 ) ) ;
#39149=CARTESIAN_POINT ( 'NONE',  ( 9.399999999999918643, 12.50000000000000000, -0.2813168883297408329 ) ) ;
#39150=ORIENTED_EDGE ( 'NONE', *, *, #79699, .T. ) ;
#39151=ORIENTED_EDGE ( 'NONE', *, *, #12716, .F. ) ;
#39152=ORIENTED_EDGE ( 'NONE', *, *, #62035, .T. ) ;
#39153=ORIENTED_EDGE ( 'NONE', *, *, #98910, .T. ) ;
#39154=DIRECTION ( 'NONE',  ( 0.000000000000000000, 1.000000000000000000, 0.000000000000000000 ) ) ;
#39155=DIRECTION ( 'NONE',  ( -4.274815082592931898E-19, -0.9999939076577903929, -0.003490651415223739937 ) ) ;
#39156=FACE_BOUND ( 'NONE', #65462, .T. ) ;
#39157=DIRECTION ( 'NONE',  ( 0.000000000000000000, 0.000000000000000000, 1.000000000000000000 ) ) ;
#39158=ADVANCED_FACE ( 'NONE', ( #81967 ), #91591, .T. ) ;
#39159=CIRCLE ( 'NONE', #41211, 0.06509327318403745899 ) ;
#39160=EDGE_LOOP ( 'NONE', ( #109608, #125160 ) ) ;
#39161=CARTESIAN_POINT ( 'NONE',  ( -6.050000000000022027, 12.50000000000000000, -6.083687093685488989 ) ) ;
#39162=DIRECTION ( 'NONE',  ( -0.000000000000000000, 1.000000000000000000, -0.000000000000000000 ) ) ;
#39163=DIRECTION ( 'NONE',  ( 0.000000000000000000, 1.000000000000000000, 0.000000000000000000 ) ) ;
#39164=DIRECTION ( 'NONE',  ( -0.000000000000000000, 1.000000000000000000, -0.000000000000000000 ) ) ;
#39165=DIRECTION ( 'NONE',  ( 0.000000000000000000, 0.000000000000000000, 1.000000000000000000 ) ) ;
#39166=EDGE_LOOP ( 'NONE', ( #15779, #1858, #109249, #70119 ) ) ;
#39167=CARTESIAN_POINT ( 'NONE',  ( 6.649999999999931966, 12.50000000000000000, -7.253104124594891289 ) ) ;
#39168=AXIS2_PLACEMENT_3D ( 'NONE', #119710, #90239, #37939 ) ;
#39169=EDGE_CURVE ( 'NONE', #77956, #33245, #112086, .T. ) ;
#39171=ORIENTED_EDGE ( 'NONE', *, *, #9630, .T. ) ;
#39172=DIRECTION ( 'NONE',  ( 0.000000000000000000, -0.000000000000000000, 1.000000000000000000 ) ) ;
#39173=CARTESIAN_POINT ( 'NONE',  ( -3.750000000000025757, 2.500000000000000000, -2.757883832488654097 ) ) ;
#39174=ORIENTED_EDGE ( 'NONE', *, *, #40725, .F. ) ;
#39175=CONICAL_SURFACE ( 'NONE', #58033, 0.1000000000000002554, 0.003490658503988666988 ) ;
#39176=VECTOR ( 'NONE', #73887, 1000.000000000000000 ) ;
#39177=VECTOR ( 'NONE', #59107, 1000.000000000000000 ) ;
#39178=CARTESIAN_POINT ( 'NONE',  ( -10.60000000000000320, 2.500000000000000000, -4.776537180435973085 ) ) ;
#39179=FACE_OUTER_BOUND ( 'NONE', #33780, .T. ) ;
#39180=VERTEX_POINT ( 'NONE', #34175 ) ;
#39181=DIRECTION ( 'NONE',  ( 0.000000000000000000, 1.000000000000000000, 0.000000000000000000 ) ) ;
#39182=EDGE_LOOP ( 'NONE', ( #69972, #58147 ) ) ;
#39183=DIRECTION ( 'NONE',  ( -4.274815082592931898E-19, -0.9999939076577903929, -0.003490651415223739937 ) ) ;
#39184=ORIENTED_EDGE ( 'NONE', *, *, #123105, .F. ) ;
#39185=CARTESIAN_POINT ( 'NONE',  ( -14.14999999999998614, 2.500000000000000000, -2.165063509461099489 ) ) ;
#39186=FACE_BOUND ( 'NONE', #107876, .T. ) ;
#39187=VECTOR ( 'NONE', #31117, 1000.000000000000000 ) ;
#39188=ORIENTED_EDGE ( 'NONE', *, *, #49773, .F. ) ;
#39190=EDGE_LOOP ( 'NONE', ( #10229, #102180 ) ) ;
#39191=CARTESIAN_POINT ( 'NONE',  ( 0.7999999999999612976, 2.500000000000000000, -0.1000000000000001166 ) ) ;
#39192=LINE ( 'NONE', #37869, #80087 ) ;
#39193=CARTESIAN_POINT ( 'NONE',  ( 9.149999999999920419, 2.500000000000000000, 2.857883832488649301 ) ) ;
#39194=PLANE ( 'NONE',  #13166 ) ;
#39195=CARTESIAN_POINT ( 'NONE',  ( -4.250072516143177381E-14, 2.500000000000000000, -3.537306695894649966 ) ) ;
#39196=AXIS2_PLACEMENT_3D ( 'NONE', #12420, #51088, #41908 ) ;
#39197=ORIENTED_EDGE ( 'NONE', *, *, #54307, .F. ) ;
#39198=CONICAL_SURFACE ( 'NONE', #5705, 0.09999999999999982514, 0.003490658503988666988 ) ;
#39199=ORIENTED_EDGE ( 'NONE', *, *, #58006, .T. ) ;
#39200=EDGE_CURVE ( 'NONE', #103444, #96136, #44630, .T. ) ;
#39201=VERTEX_POINT ( 'NONE', #5335 ) ;
#39202=DIRECTION ( 'NONE',  ( -0.000000000000000000, -1.000000000000000000, -0.000000000000000000 ) ) ;
#39203=CIRCLE ( 'NONE', #37130, 0.06509327318403745899 ) ;
#39204=CARTESIAN_POINT ( 'NONE',  ( -1.650000000000034772, 2.500000000000000000, 6.495190528383297135 ) ) ;
#39206=VERTEX_POINT ( 'NONE', #55732 ) ;
#39207=ORIENTED_EDGE ( 'NONE', *, *, #118387, .F. ) ;
#39208=ORIENTED_EDGE ( 'NONE', *, *, #74520, .T. ) ;
#39209=DIRECTION ( 'NONE',  ( 0.000000000000000000, 0.000000000000000000, 1.000000000000000000 ) ) ;
#39210=CIRCLE ( 'NONE', #43404, 0.06509327318403745899 ) ;
#39211=AXIS2_PLACEMENT_3D ( 'NONE', #43033, #72473, #63935 ) ;
#39213=EDGE_CURVE ( 'NONE', #16894, #102223, #46546, .T. ) ;
#39214=AXIS2_PLACEMENT_3D ( 'NONE', #83823, #75296, #22992 ) ;
#39216=LINE ( 'NONE', #79751, #63640 ) ;
#39217=LINE ( 'NONE', #120328, #4316 ) ;
#39218=CARTESIAN_POINT ( 'NONE',  ( -5.800000000000018474, 12.50000000000000000, 4.330127018922196314 ) ) ;
#39219=DIRECTION ( 'NONE',  ( -0.000000000000000000, 1.000000000000000000, -0.000000000000000000 ) ) ;
#39220=CARTESIAN_POINT ( 'NONE',  ( -10.65000000000000213, 2.500000000000000000, 2.511473670974873507 ) ) ;
#39221=ADVANCED_FACE ( 'NONE', ( #17058 ), #85325, .T. ) ;
#39222=AXIS2_PLACEMENT_3D ( 'NONE', #81667, #32606, #22775 ) ;
#39223=EDGE_CURVE ( 'NONE', #4340, #48111, #102061, .T. ) ;
#39224=DIRECTION ( 'NONE',  ( -4.274815082592931898E-19, -0.9999939076577903929, -0.003490651415223739937 ) ) ;
#39225=VERTEX_POINT ( 'NONE', #76018 ) ;
#39226=ORIENTED_EDGE ( 'NONE', *, *, #98224, .T. ) ;
#39227=DIRECTION ( 'NONE',  ( -0.000000000000000000, -1.000000000000000000, -0.000000000000000000 ) ) ;
#39228=AXIS2_PLACEMENT_3D ( 'NONE', #99084, #38901, #38233 ) ;
#39229=CIRCLE ( 'NONE', #112353, 0.1000000000000000472 ) ;
#39230=EDGE_CURVE ( 'NONE', #114770, #128977, #64396, .T. ) ;
#39232=ORIENTED_EDGE ( 'NONE', *, *, #24573, .T. ) ;
#39234=ADVANCED_FACE ( 'NONE', ( #106125 ), #22653, .T. ) ;
#39236=CARTESIAN_POINT ( 'NONE',  ( -1.850000000000033396, 12.50000000000000000, -6.213873640053564351 ) ) ;
#39237=CARTESIAN_POINT ( 'NONE',  ( 12.89999999999990266, 2.500000000000000000, -4.922947341949753586 ) ) ;
#39238=CARTESIAN_POINT ( 'NONE',  ( 13.09999999999990195, 12.50000000000000000, 4.611443907251934426 ) ) ;
#39239=DIRECTION ( 'NONE',  ( -0.000000000000000000, 1.000000000000000000, -0.000000000000000000 ) ) ;
#39240=DIRECTION ( 'NONE',  ( 0.000000000000000000, -0.9999939076577903929, 0.003490651415223739937 ) ) ;
#39241=DIRECTION ( 'NONE',  ( -0.000000000000000000, 1.000000000000000000, -0.000000000000000000 ) ) ;
#39242=CONICAL_SURFACE ( 'NONE', #103964, 0.1000000000000002554, 0.003490658503988666988 ) ;
#39243=CARTESIAN_POINT ( 'NONE',  ( 7.049999999999928768, 12.50000000000000000, -2.230156782645139391 ) ) ;
#39244=ORIENTED_EDGE ( 'NONE', *, *, #7266, .F. ) ;
#39245=EDGE_CURVE ( 'NONE', #83964, #118566, #81137, .T. ) ;
#39246=VERTEX_POINT ( 'NONE', #57007 ) ;
#39247=ORIENTED_EDGE ( 'NONE', *, *, #69082, .F. ) ;
#39248=ORIENTED_EDGE ( 'NONE', *, *, #108929, .T. ) ;
#39249=DIRECTION ( 'NONE',  ( 0.000000000000000000, 0.000000000000000000, 1.000000000000000000 ) ) ;
#39250=DIRECTION ( 'NONE',  ( 0.000000000000000000, 1.000000000000000000, 0.000000000000000000 ) ) ;
#39251=VERTEX_POINT ( 'NONE', #85825 ) ;
#39252=VECTOR ( 'NONE', #200, 1000.000000000000000 ) ;
#39253=DIRECTION ( 'NONE',  ( 0.000000000000000000, 1.000000000000000000, 0.000000000000000000 ) ) ;
#39254=EDGE_CURVE ( 'NONE', #40453, #21310, #78809, .T. ) ;
#39255=AXIS2_PLACEMENT_3D ( 'NONE', #84638, #55820, #124571 ) ;
#39256=CARTESIAN_POINT ( 'NONE',  ( 8.949999999999919353, 12.50000000000000000, -6.148780366869526226 ) ) ;
#39257=CARTESIAN_POINT ( 'NONE',  ( 8.749999999999953815, 2.500000000000000000, -2.065063509461102065 ) ) ;
#39258=LINE ( 'NONE', #78532, #53804 ) ;
#39259=EDGE_LOOP ( 'NONE', ( #66108, #82113 ) ) ;
#39260=CARTESIAN_POINT ( 'NONE',  ( 11.24999999999990941, 12.50000000000000000, 7.122917578226811486 ) ) ;
#39261=CIRCLE ( 'NONE', #37190, 0.1000000000000002554 ) ;
#39262=EDGE_CURVE ( 'NONE', #104716, #71809, #112243, .T. ) ;
#39263=DIRECTION ( 'NONE',  ( 0.000000000000000000, -0.000000000000000000, 1.000000000000000000 ) ) ;
#39264=EDGE_LOOP ( 'NONE', ( #71280, #43727 ) ) ;
#39265=AXIS2_PLACEMENT_3D ( 'NONE', #103583, #96312, #85213 ) ;
#39266=AXIS2_PLACEMENT_3D ( 'NONE', #78557, #89007, #18950 ) ;
#39267=ORIENTED_EDGE ( 'NONE', *, *, #87473, .T. ) ;
#39268=ORIENTED_EDGE ( 'NONE', *, *, #30790, .T. ) ;
#39269=ORIENTED_EDGE ( 'NONE', *, *, #63436, .T. ) ;
#39270=CARTESIAN_POINT ( 'NONE',  ( 9.599999999999914380, 2.500000000000000000, -3.737306695894649700 ) ) ;
#39271=ADVANCED_FACE ( 'NONE', ( #55095 ), #108305, .T. ) ;
#39272=EDGE_CURVE ( 'NONE', #83854, #63832, #14211, .T. ) ;
#39273=EDGE_CURVE ( 'NONE', #2826, #55428, #39394, .T. ) ;
#39274=CARTESIAN_POINT ( 'NONE',  ( -8.350000000000013856, 12.50000000000000000, -5.867463478539781896 ) ) ;
#39275=FACE_OUTER_BOUND ( 'NONE', #38767, .T. ) ;
#39276=VECTOR ( 'NONE', #66174, 1000.000000000000000 ) ;
#39277=EDGE_CURVE ( 'NONE', #65565, #74025, #74736, .T. ) ;
#39278=VERTEX_POINT ( 'NONE', #116577 ) ;
#39279=CONICAL_SURFACE ( 'NONE', #74941, 0.1000000000000002554, 0.003490658503988666988 ) ;
#39280=DIRECTION ( 'NONE',  ( 0.000000000000000000, 0.000000000000000000, 1.000000000000000000 ) ) ;
#39281=DIRECTION ( 'NONE',  ( 0.000000000000000000, 1.000000000000000000, 0.000000000000000000 ) ) ;
#39282=CARTESIAN_POINT ( 'NONE',  ( 3.749999999999942268, 12.50000000000000000, 1.472243186433545459 ) ) ;
#39283=DIRECTION ( 'NONE',  ( 0.000000000000000000, -0.9999939076577903929, 0.003490651415223739937 ) ) ;
#39284=EDGE_CURVE ( 'NONE', #5464, #93629, #95514, .T. ) ;
#39285=EDGE_CURVE ( 'NONE', #37787, #112012, #91306, .T. ) ;
#39286=ORIENTED_EDGE ( 'NONE', *, *, #113132, .F. ) ;
#39287=AXIS2_PLACEMENT_3D ( 'NONE', #125546, #16852, #56157 ) ;
#39288=ADVANCED_FACE ( 'NONE', ( #117197 ), #124756, .T. ) ;
#39289=CARTESIAN_POINT ( 'NONE',  ( 1.649999999999951505, 2.500000000000000000, -2.957883832488653830 ) ) ;
#39290=CONICAL_SURFACE ( 'NONE', #26644, 0.1000000000000000472, 0.003490658503988666988 ) ;
#39291=ORIENTED_EDGE ( 'NONE', *, *, #5681, .F. ) ;
#39292=VERTEX_POINT ( 'NONE', #85193 ) ;
#39293=CARTESIAN_POINT ( 'NONE',  ( 8.749999999999953815, 2.500000000000000000, 6.495190528383297135 ) ) ;
#39294=CARTESIAN_POINT ( 'NONE',  ( 8.099999999999921485, 2.500000000000000000, 0.3464101615137735735 ) ) ;
#39295=FACE_BOUND ( 'NONE', #11858, .T. ) ;
#39296=VECTOR ( 'NONE', #61387, 1000.000000000000000 ) ;
#39297=CARTESIAN_POINT ( 'NONE',  ( -5.850000000000022737, 12.50000000000000000, -2.165063509461101710 ) ) ;
#39298=DIRECTION ( 'NONE',  ( 0.000000000000000000, 0.000000000000000000, 1.000000000000000000 ) ) ;
#39299=AXIS2_PLACEMENT_3D ( 'NONE', #91018, #41287, #94230 ) ;
#39300=CARTESIAN_POINT ( 'NONE',  ( 13.94999999999989448, 12.50000000000000000, -2.511473670974877948 ) ) ;
#39301=ORIENTED_EDGE ( 'NONE', *, *, #36899, .F. ) ;
#39302=CARTESIAN_POINT ( 'NONE',  ( -6.450000000000014388, 2.500000000000000000, 1.918653347947321564 ) ) ;
#39303=DIRECTION ( 'NONE',  ( 0.000000000000000000, 0.000000000000000000, -1.000000000000000000 ) ) ;
#39304=CIRCLE ( 'NONE', #66445, 0.09999999999999982514 ) ;
#39305=CARTESIAN_POINT ( 'NONE',  ( 0.7999999999999553024, 12.50000000000000000, -4.395220292106239768 ) ) ;
#39306=DIRECTION ( 'NONE',  ( -0.000000000000000000, 1.000000000000000000, -0.000000000000000000 ) ) ;
#39307=ORIENTED_EDGE ( 'NONE', *, *, #108221, .F. ) ;
#39308=LINE ( 'NONE', #118467, #78374 ) ;
#39309=AXIS2_PLACEMENT_3D ( 'NONE', #122647, #32995, #23810 ) ;
#39311=ORIENTED_EDGE ( 'NONE', *, *, #5565, .F. ) ;
#39312=VERTEX_POINT ( 'NONE', #35464 ) ;
#39313=CARTESIAN_POINT ( 'NONE',  ( -5.850000000000021849, 2.500000000000000000, -1.572243186433550211 ) ) ;
#39314=CONICAL_SURFACE ( 'NONE', #101983, 0.1000000000000002554, 0.003490658503988666988 ) ;
#39315=DIRECTION ( 'NONE',  ( 0.000000000000000000, 0.000000000000000000, 1.000000000000000000 ) ) ;
#39316=FACE_BOUND ( 'NONE', #69853, .T. ) ;
#39317=DIRECTION ( 'NONE',  ( 0.000000000000000000, 0.000000000000000000, 1.000000000000000000 ) ) ;
#39318=AXIS2_PLACEMENT_3D ( 'NONE', #85858, #84593, #96323 ) ;
#39319=AXIS2_PLACEMENT_3D ( 'NONE', #116036, #86568, #47953 ) ;
#39320=CARTESIAN_POINT ( 'NONE',  ( 12.89999999999990088, 2.500000000000000000, 4.330127018922196314 ) ) ;
#39321=ORIENTED_EDGE ( 'NONE', *, *, #129357, .T. ) ;
#39322=DIRECTION ( 'NONE',  ( -4.274815082592931898E-19, -0.9999939076577903929, -0.003490651415223739937 ) ) ;
#39325=CARTESIAN_POINT ( 'NONE',  ( -0.6000000000000323963, 2.500000000000000000, 0.3464101615137759604 ) ) ;
#39326=DIRECTION ( 'NONE',  ( -0.000000000000000000, -1.000000000000000000, -0.000000000000000000 ) ) ;
#39328=DIRECTION ( 'NONE',  ( 0.000000000000000000, 0.000000000000000000, 1.000000000000000000 ) ) ;
#39329=CARTESIAN_POINT ( 'NONE',  ( -6.450000000000017941, 2.500000000000000000, -2.411473670974877859 ) ) ;
#39330=ORIENTED_EDGE ( 'NONE', *, *, #86694, .F. ) ;
#39331=DIRECTION ( 'NONE',  ( -0.000000000000000000, 1.000000000000000000, -0.000000000000000000 ) ) ;
#39333=CARTESIAN_POINT ( 'NONE',  ( 3.299999999999944755, 2.500000000000000000, -4.230127018922201998 ) ) ;
#39334=ORIENTED_EDGE ( 'NONE', *, *, #71830, .T. ) ;
#39336=EDGE_LOOP ( 'NONE', ( #69360, #127861 ) ) ;
#39337=CARTESIAN_POINT ( 'NONE',  ( 17.99892160975036859, 2.500000000000000444, 4.934975027008750459 ) ) ;
#39338=ORIENTED_EDGE ( 'NONE', *, *, #63545, .F. ) ;
#39339=CARTESIAN_POINT ( 'NONE',  ( 10.79999999999991367, 2.500000000000000000, -2.385244779468109755E-15 ) ) ;
#39340=CARTESIAN_POINT ( 'NONE',  ( 2.899999999999944844, 12.50000000000000000, 5.022947341949748790 ) ) ;
#39341=AXIS2_PLACEMENT_3D ( 'NONE', #28891, #17758, #57706 ) ;
#39342=LINE ( 'NONE', #31284, #43072 ) ;
#39343=CIRCLE ( 'NONE', #91548, 0.06509327318403745899 ) ;
#39344=CARTESIAN_POINT ( 'NONE',  ( 9.999999999999911182, 2.500000000000000000, 4.922947341949748257 ) ) ;
#39346=DIRECTION ( 'NONE',  ( -0.000000000000000000, 1.000000000000000000, -0.000000000000000000 ) ) ;
#39347=DIRECTION ( 'NONE',  ( 0.000000000000000000, 0.000000000000000000, 1.000000000000000000 ) ) ;
#39348=LINE ( 'NONE', #8545, #77832 ) ;
#39351=LINE ( 'NONE', #56375, #70255 ) ;
#39352=AXIS2_PLACEMENT_3D ( 'NONE', #75559, #97789, #67017 ) ;
#39353=ORIENTED_EDGE ( 'NONE', *, *, #1700, .T. ) ;
#39354=AXIS2_PLACEMENT_3D ( 'NONE', #11724, #52302, #11065 ) ;
#39355=ORIENTED_EDGE ( 'NONE', *, *, #98930, .F. ) ;
#39356=DIRECTION ( 'NONE',  ( -0.000000000000000000, 1.000000000000000000, -0.000000000000000000 ) ) ;
#39357=VERTEX_POINT ( 'NONE', #119163 ) ;
#39358=CARTESIAN_POINT ( 'NONE',  ( 7.299999999999926104, 2.500000000000000000, 4.576537180435972019 ) ) ;
#39359=ORIENTED_EDGE ( 'NONE', *, *, #125053, .T. ) ;
#39360=VERTEX_POINT ( 'NONE', #77947 ) ;
#39361=ORIENTED_EDGE ( 'NONE', *, *, #7266, .T. ) ;
#39362=CARTESIAN_POINT ( 'NONE',  ( -12.04999999999999716, 12.50000000000000000, -6.495190528383298911 ) ) ;
#39363=CIRCLE ( 'NONE', #10090, 0.1000000000000002554 ) ;
#39364=FACE_OUTER_BOUND ( 'NONE', #112594, .T. ) ;
#39366=CARTESIAN_POINT ( 'NONE',  ( -3.150000000000033218, 12.50000000000000000, -6.906693963081115939 ) ) ;
#39367=PLANE ( 'NONE',  #82807 ) ;
#39368=FACE_OUTER_BOUND ( 'NONE', #99552, .T. ) ;
#39369=CARTESIAN_POINT ( 'NONE',  ( 2.949999999999946887, 2.500000000000000000, -2.265063509461101798 ) ) ;
#39370=CONICAL_SURFACE ( 'NONE', #20562, 0.1000000000000002554, 0.003490658503988666988 ) ;
#39371=FACE_OUTER_BOUND ( 'NONE', #92871, .T. ) ;
#39372=EDGE_CURVE ( 'NONE', #77356, #20308, #20326, .T. ) ;
#39373=EDGE_CURVE ( 'NONE', #8757, #50689, #97837, .T. ) ;
#39374=DIRECTION ( 'NONE',  ( -0.000000000000000000, 1.000000000000000000, -0.000000000000000000 ) ) ;
#39375=ORIENTED_EDGE ( 'NONE', *, *, #99731, .F. ) ;
#39376=CIRCLE ( 'NONE', #12233, 0.06509327318403745899 ) ;
#39377=ORIENTED_EDGE ( 'NONE', *, *, #7076, .T. ) ;
#39379=EDGE_CURVE ( 'NONE', #60176, #31905, #41445, .T. ) ;
#39380=CARTESIAN_POINT ( 'NONE',  ( 6.849999999999929479, 2.500000000000000000, 6.048780366869520364 ) ) ;
#39381=EDGE_CURVE ( 'NONE', #109510, #44029, #58157, .T. ) ;
#39382=ORIENTED_EDGE ( 'NONE', *, *, #70730, .F. ) ;
#39383=ORIENTED_EDGE ( 'NONE', *, *, #60253, .T. ) ;
#39384=EDGE_CURVE ( 'NONE', #90957, #24019, #49554, .T. ) ;
#39385=DIRECTION ( 'NONE',  ( 0.000000000000000000, 0.000000000000000000, 1.000000000000000000 ) ) ;
#39386=AXIS2_PLACEMENT_3D ( 'NONE', #36929, #67654, #96461 ) ;
#39387=AXIS2_PLACEMENT_3D ( 'NONE', #37262, #71061, #1661 ) ;
#39388=CARTESIAN_POINT ( 'NONE',  ( 11.84999999999990372, 12.50000000000000000, -6.841600689897078702 ) ) ;
#39389=CONICAL_SURFACE ( 'NONE', #95789, 0.1000000000000002554, 0.003490658503988666988 ) ;
#39390=DIRECTION ( 'NONE',  ( 0.000000000000000000, 1.000000000000000000, 0.000000000000000000 ) ) ;
#39391=LINE ( 'NONE', #30205, #117983 ) ;
#39392=FACE_OUTER_BOUND ( 'NONE', #9639, .T. ) ;
#39393=VERTEX_POINT ( 'NONE', #120454 ) ;
#39394=CIRCLE ( 'NONE', #112533, 0.1000000000000002554 ) ;
#39395=ORIENTED_EDGE ( 'NONE', *, *, #34481, .F. ) ;
#39396=CARTESIAN_POINT ( 'NONE',  ( 7.299999999999926104, 2.500000000000000000, -3.983716857408426293 ) ) ;
#39397=ORIENTED_EDGE ( 'NONE', *, *, #39097, .T. ) ;
#39398=DIRECTION ( 'NONE',  ( 0.000000000000000000, 0.000000000000000000, 1.000000000000000000 ) ) ;
#39399=ORIENTED_EDGE ( 'NONE', *, *, #59804, .T. ) ;
#39400=AXIS2_PLACEMENT_3D ( 'NONE', #48963, #108505, #76486 ) ;
#39401=ORIENTED_EDGE ( 'NONE', *, *, #64829, .F. ) ;
#39402=FACE_OUTER_BOUND ( 'NONE', #46947, .T. ) ;
#39403=DIRECTION ( 'NONE',  ( 0.000000000000000000, 1.000000000000000000, 0.000000000000000000 ) ) ;
#39404=AXIS2_PLACEMENT_3D ( 'NONE', #77989, #77348, #111133 ) ;
#39405=AXIS2_PLACEMENT_3D ( 'NONE', #98315, #9304, #29587 ) ;
#39406=CARTESIAN_POINT ( 'NONE',  ( 8.099999999999921485, 2.500000000000000000, -0.3464101615137783474 ) ) ;
#39407=FACE_OUTER_BOUND ( 'NONE', #43856, .T. ) ;
#39408=DIRECTION ( 'NONE',  ( -0.000000000000000000, -1.000000000000000000, -0.000000000000000000 ) ) ;
#39409=VERTEX_POINT ( 'NONE', #59629 ) ;
#39410=DIRECTION ( 'NONE',  ( 0.000000000000000000, -0.000000000000000000, 1.000000000000000000 ) ) ;
#39411=LINE ( 'NONE', #79327, #103809 ) ;
#39412=DIRECTION ( 'NONE',  ( -0.000000000000000000, -1.000000000000000000, -0.000000000000000000 ) ) ;
#39413=DIRECTION ( 'NONE',  ( 0.000000000000000000, 0.000000000000000000, -1.000000000000000000 ) ) ;
#39414=DIRECTION ( 'NONE',  ( -0.000000000000000000, -1.000000000000000000, -0.000000000000000000 ) ) ;
#39415=VERTEX_POINT ( 'NONE', #60274 ) ;
#39416=ORIENTED_EDGE ( 'NONE', *, *, #13023, .T. ) ;
#39417=ADVANCED_FACE ( 'NONE', ( #69407 ), #11972, .T. ) ;
#39418=AXIS2_PLACEMENT_3D ( 'NONE', #41392, #50535, #19807 ) ;
#39419=CARTESIAN_POINT ( 'NONE',  ( -10.00000000000000711, 2.500000000000000000, -3.637306695894645614 ) ) ;
#39420=EDGE_CURVE ( 'NONE', #80133, #104306, #50420, .T. ) ;
#39421=EDGE_CURVE ( 'NONE', #76087, #126646, #99539, .T. ) ;
#39422=ORIENTED_EDGE ( 'NONE', *, *, #85776, .T. ) ;
#39423=FACE_OUTER_BOUND ( 'NONE', #122819, .T. ) ;
#39424=CARTESIAN_POINT ( 'NONE',  ( 4.199999999999941558, 12.50000000000000000, -4.330127018922201643 ) ) ;
#39425=AXIS2_PLACEMENT_3D ( 'NONE', #60950, #10549, #50490 ) ;
#39426=CIRCLE ( 'NONE', #62398, 0.1000000000000002554 ) ;
#39427=CIRCLE ( 'NONE', #56109, 0.06509327318403745899 ) ;
#39428=EDGE_CURVE ( 'NONE', #98725, #63253, #89703, .T. ) ;
#39429=EDGE_LOOP ( 'NONE', ( #44876, #78237 ) ) ;
#39430=CARTESIAN_POINT ( 'NONE',  ( -8.150000000000012790, 2.500000000000000000, 1.718653347947321386 ) ) ;
#39432=EDGE_CURVE ( 'NONE', #32314, #40954, #28714, .T. ) ;
#39433=DIRECTION ( 'NONE',  ( 0.000000000000000000, 1.000000000000000000, 0.000000000000000000 ) ) ;
#39434=DIRECTION ( 'NONE',  ( 0.000000000000000000, 1.000000000000000000, 0.000000000000000000 ) ) ;
#39435=EDGE_LOOP ( 'NONE', ( #73611, #83852, #113308, #19327 ) ) ;
#39436=EDGE_CURVE ( 'NONE', #60183, #122361, #30779, .T. ) ;
#39437=EDGE_CURVE ( 'NONE', #79801, #105776, #87757, .T. ) ;
#39438=AXIS2_PLACEMENT_3D ( 'NONE', #3132, #82345, #102602 ) ;
#39439=EDGE_CURVE ( 'NONE', #60348, #4520, #118513, .T. ) ;
#39440=CARTESIAN_POINT ( 'NONE',  ( 3.099999999999945022, 2.500000000000000000, -0.2464101615137783419 ) ) ;
#39442=CARTESIAN_POINT ( 'NONE',  ( 48.84099803997424516, 2.320797884491624163, -5.300800515398695012 ) ) ;
#39443=DIRECTION ( 'NONE',  ( 0.000000000000000000, 1.000000000000000000, 0.000000000000000000 ) ) ;
#39444=ADVANCED_FACE ( 'NONE', ( #20963 ), #129085, .T. ) ;
#39445=AXIS2_PLACEMENT_3D ( 'NONE', #105262, #15579, #125541 ) ;
#39446=DIRECTION ( 'NONE',  ( 0.000000000000000000, -0.9999939076577903929, 0.003490651415223739937 ) ) ;
#39447=AXIS2_PLACEMENT_3D ( 'NONE', #84457, #34735, #66092 ) ;
#39448=ORIENTED_EDGE ( 'NONE', *, *, #11430, .F. ) ;
#39449=LINE ( 'NONE', #113147, #99141 ) ;
#39450=ORIENTED_EDGE ( 'NONE', *, *, #115091, .F. ) ;
#39451=DIRECTION ( 'NONE',  ( -0.000000000000000000, -1.000000000000000000, -0.000000000000000000 ) ) ;
#39452=DIRECTION ( 'NONE',  ( -0.000000000000000000, 1.000000000000000000, -0.000000000000000000 ) ) ;
#39453=PLANE ( 'NONE',  #102045 ) ;
#39454=ORIENTED_EDGE ( 'NONE', *, *, #53008, .T. ) ;
#39455=AXIS2_PLACEMENT_3D ( 'NONE', #32581, #106288, #16602 ) ;
#39456=DIRECTION ( 'NONE',  ( 0.000000000000000000, -0.000000000000000000, 1.000000000000000000 ) ) ;
#39457=DIRECTION ( 'NONE',  ( -0.000000000000000000, 1.000000000000000000, -0.000000000000000000 ) ) ;
#39458=AXIS2_PLACEMENT_3D ( 'NONE', #98375, #128530, #59787 ) ;
#39459=VECTOR ( 'NONE', #116317, 1000.000000000000000 ) ;
#39460=ORIENTED_EDGE ( 'NONE', *, *, #74509, .F. ) ;
#39461=DIRECTION ( 'NONE',  ( 0.000000000000000000, 1.000000000000000000, 0.000000000000000000 ) ) ;
#39462=ORIENTED_EDGE ( 'NONE', *, *, #82965, .T. ) ;
#39463=DIRECTION ( 'NONE',  ( -0.000000000000000000, -1.000000000000000000, -0.000000000000000000 ) ) ;
#39464=CIRCLE ( 'NONE', #56146, 0.06509327318403743123 ) ;
#39465=ORIENTED_EDGE ( 'NONE', *, *, #19389, .F. ) ;
#39466=DIRECTION ( 'NONE',  ( 0.000000000000000000, 0.000000000000000000, 1.000000000000000000 ) ) ;
#39467=CARTESIAN_POINT ( 'NONE',  ( 13.39473262249372176, 2.500000000000001332, -7.044698190877980437 ) ) ;
#39468=ORIENTED_EDGE ( 'NONE', *, *, #35024, .T. ) ;
#39469=EDGE_LOOP ( 'NONE', ( #60884, #6818, #107456, #112254 ) ) ;
#39470=FACE_OUTER_BOUND ( 'NONE', #48032, .T. ) ;
#39471=DIRECTION ( 'NONE',  ( 0.000000000000000000, 0.000000000000000000, 1.000000000000000000 ) ) ;
#39472=ORIENTED_EDGE ( 'NONE', *, *, #2360, .T. ) ;
#39475=CIRCLE ( 'NONE', #79177, 0.06509327318403745899 ) ;
#39476=EDGE_CURVE ( 'NONE', #106311, #25426, #74670, .T. ) ;
#39477=DIRECTION ( 'NONE',  ( 0.000000000000000000, 0.000000000000000000, -1.000000000000000000 ) ) ;
#39478=DIRECTION ( 'NONE',  ( 0.000000000000000000, 0.000000000000000000, 1.000000000000000000 ) ) ;
#39480=DIRECTION ( 'NONE',  ( 0.000000000000000000, 0.000000000000000000, -1.000000000000000000 ) ) ;
#39481=DIRECTION ( 'NONE',  ( -0.000000000000000000, 1.000000000000000000, -0.000000000000000000 ) ) ;
#39482=AXIS2_PLACEMENT_3D ( 'NONE', #51874, #53162, #84544 ) ;
#39483=VERTEX_POINT ( 'NONE', #58331 ) ;
#39484=ORIENTED_EDGE ( 'NONE', *, *, #40082, .T. ) ;
#39485=AXIS2_PLACEMENT_3D ( 'NONE', #74674, #3986, #104137 ) ;
#39486=ORIENTED_EDGE ( 'NONE', *, *, #18579, .F. ) ;
#39487=EDGE_LOOP ( 'NONE', ( #119936, #27384 ) ) ;
#39488=DIRECTION ( 'NONE',  ( -0.000000000000000000, -1.000000000000000000, -0.000000000000000000 ) ) ;
#39489=CARTESIAN_POINT ( 'NONE',  ( -5.600000000000020073, 2.500000000000000000, 0.4464101615137736623 ) ) ;
#39490=DIRECTION ( 'NONE',  ( -0.000000000000000000, -1.000000000000000000, -0.000000000000000000 ) ) ;
#39491=AXIS2_PLACEMENT_3D ( 'NONE', #107717, #75661, #107056 ) ;
#39492=ORIENTED_EDGE ( 'NONE', *, *, #20354, .F. ) ;
#39493=ADVANCED_FACE ( 'NONE', ( #58962 ), #16155, .T. ) ;
#39494=FACE_BOUND ( 'NONE', #14072, .T. ) ;
#39496=DIRECTION ( 'NONE',  ( 0.000000000000000000, 0.000000000000000000, 1.000000000000000000 ) ) ;
#39497=DIRECTION ( 'NONE',  ( 0.000000000000000000, 1.000000000000000000, 0.000000000000000000 ) ) ;
#39498=DIRECTION ( 'NONE',  ( 0.000000000000000000, 0.000000000000000000, 1.000000000000000000 ) ) ;
#39499=VECTOR ( 'NONE', #75102, 1000.000000000000000 ) ;
#39500=AXIS2_PLACEMENT_3D ( 'NONE', #5736, #18147, #97358 ) ;
#39501=CARTESIAN_POINT ( 'NONE',  ( -9.150000000000009237, 12.50000000000000000, -2.857883832488653741 ) ) ;
#39502=DIRECTION ( 'NONE',  ( -4.274815082592931898E-19, -0.9999939076577903929, -0.003490651415223739937 ) ) ;
#39503=DIRECTION ( 'NONE',  ( 0.000000000000000000, 0.000000000000000000, 1.000000000000000000 ) ) ;
#39504=DIRECTION ( 'NONE',  ( 0.000000000000000000, -0.9999939076577903929, 0.003490651415223739937 ) ) ;
#39505=CARTESIAN_POINT ( 'NONE',  ( -6.450000000000016165, 12.50000000000000000, 6.906693963081109722 ) ) ;
#39506=DIRECTION ( 'NONE',  ( 0.000000000000000000, -0.9999939076577903929, 0.003490651415223739937 ) ) ;
#39507=CARTESIAN_POINT ( 'NONE',  ( -12.29999999999999716, 12.50000000000000000, -3.918623584224386391 ) ) ;
#39508=ORIENTED_EDGE ( 'NONE', *, *, #104290, .F. ) ;
#39509=ORIENTED_EDGE ( 'NONE', *, *, #49919, .T. ) ;
#39510=ORIENTED_EDGE ( 'NONE', *, *, #118436, .F. ) ;
#39511=VERTEX_POINT ( 'NONE', #49160 ) ;
#39512=CARTESIAN_POINT ( 'NONE',  ( -14.34999999999998543, 2.500000000000000000, 2.611473670974877148 ) ) ;
#39513=CIRCLE ( 'NONE', #106373, 0.1000000000000002554 ) ;
#39514=LINE ( 'NONE', #116107, #29730 ) ;
#39515=VERTEX_POINT ( 'NONE', #89068 ) ;
#39516=VERTEX_POINT ( 'NONE', #82478 ) ;
#39517=VERTEX_POINT ( 'NONE', #111249 ) ;
#39519=AXIS2_PLACEMENT_3D ( 'NONE', #96199, #66104, #15041 ) ;
#39520=EDGE_CURVE ( 'NONE', #59400, #84082, #101865, .T. ) ;
#39521=VECTOR ( 'NONE', #68983, 1000.000000000000000 ) ;
#39522=CARTESIAN_POINT ( 'NONE',  ( -10.40000000000000213, 12.50000000000000000, 0.6928203230275494784 ) ) ;
#39523=DIRECTION ( 'NONE',  ( -4.274815082592931898E-19, -0.9999939076577903929, -0.003490651415223739937 ) ) ;
#39524=DIRECTION ( 'NONE',  ( 0.000000000000000000, 1.000000000000000000, 0.000000000000000000 ) ) ;
#39525=CARTESIAN_POINT ( 'NONE',  ( -12.69999999999999218, 2.500000000000000000, 4.676537180435972552 ) ) ;
#39526=FACE_OUTER_BOUND ( 'NONE', #128010, .T. ) ;
#39527=CARTESIAN_POINT ( 'NONE',  ( 5.849999999999933031, 12.50000000000000000, 7.188010851410848723 ) ) ;
#39528=ORIENTED_EDGE ( 'NONE', *, *, #89731, .F. ) ;
#39530=VECTOR ( 'NONE', #89287, 1000.000000000000000 ) ;
#39531=CARTESIAN_POINT ( 'NONE',  ( 9.349999999999916156, 12.50000000000000000, -2.511473670974877948 ) ) ;
#39532=EDGE_LOOP ( 'NONE', ( #45857, #104906, #91956, #2609 ) ) ;
#39533=AXIS2_PLACEMENT_3D ( 'NONE', #49511, #89417, #128055 ) ;
#39534=ORIENTED_EDGE ( 'NONE', *, *, #125477, .T. ) ;
#39535=ORIENTED_EDGE ( 'NONE', *, *, #90200, .F. ) ;
#39536=ADVANCED_FACE ( 'NONE', ( #62197 ), #76734, .T. ) ;
#39537=DIRECTION ( 'NONE',  ( 0.000000000000000000, 1.000000000000000000, 0.000000000000000000 ) ) ;
#39538=EDGE_CURVE ( 'NONE', #96060, #36724, #37025, .T. ) ;
#39539=EDGE_CURVE ( 'NONE', #81272, #14213, #118577, .T. ) ;
#39541=EDGE_CURVE ( 'NONE', #119696, #17553, #57956, .T. ) ;
#39542=ADVANCED_FACE ( 'NONE', ( #42560 ), #41270, .T. ) ;
#39543=ORIENTED_EDGE ( 'NONE', *, *, #83850, .T. ) ;
#39544=CONICAL_SURFACE ( 'NONE', #83346, 0.1000000000000002554, 0.003490658503988666988 ) ;
#39545=FACE_OUTER_BOUND ( 'NONE', #63736, .T. ) ;
#39547=DIRECTION ( 'NONE',  ( 0.000000000000000000, 0.000000000000000000, -1.000000000000000000 ) ) ;
#39548=CARTESIAN_POINT ( 'NONE',  ( -9.350000000000006750, 2.500000000000000000, 1.818653347947321475 ) ) ;
#39549=DIRECTION ( 'NONE',  ( 0.000000000000000000, 0.000000000000000000, 1.000000000000000000 ) ) ;
#39550=CARTESIAN_POINT ( 'NONE',  ( 13.29999999999990301, 2.500000000000000000, 4.330127018922196314 ) ) ;
#39551=ADVANCED_FACE ( 'NONE', ( #121731 ), #80941, .T. ) ;
#39552=VERTEX_POINT ( 'NONE', #71336 ) ;
#39553=DIRECTION ( 'NONE',  ( 0.000000000000000000, 1.000000000000000000, 0.000000000000000000 ) ) ;
#39554=AXIS2_PLACEMENT_3D ( 'NONE', #62022, #82311, #114811 ) ;
#39555=ADVANCED_FACE ( 'NONE', ( #102107 ), #24502, .T. ) ;
#39556=EDGE_LOOP ( 'NONE', ( #17391, #21512, #122231, #90324 ) ) ;
#39557=CARTESIAN_POINT ( 'NONE',  ( -2.500000000000032863, 2.500000000000000000, 5.022947341949748790 ) ) ;
#39558=ORIENTED_EDGE ( 'NONE', *, *, #52106, .T. ) ;
#39559=CARTESIAN_POINT ( 'NONE',  ( 1.699999999999950218, 12.50000000000000000, 4.265033745738159077 ) ) ;
#39560=LINE ( 'NONE', #107621, #47002 ) ;
#39561=VERTEX_POINT ( 'NONE', #113862 ) ;
#39563=LINE ( 'NONE', #10683, #54063 ) ;
#39565=AXIS2_PLACEMENT_3D ( 'NONE', #40349, #48219, #28584 ) ;
#39566=CARTESIAN_POINT ( 'NONE',  ( -7.300000000000018474, 2.500000000000000000, -3.983716857408426293 ) ) ;
#39568=VERTEX_POINT ( 'NONE', #32093 ) ;
#39569=CARTESIAN_POINT ( 'NONE',  ( -6.850000000000017408, 2.500000000000000000, -2.511473670974877948 ) ) ;
#39571=DIRECTION ( 'NONE',  ( 0.000000000000000000, 0.000000000000000000, 1.000000000000000000 ) ) ;
#39572=DIRECTION ( 'NONE',  ( -4.274815082592931898E-19, -0.9999939076577903929, -0.003490651415223739937 ) ) ;
#39573=CONICAL_SURFACE ( 'NONE', #6066, 0.1000000000000002554, 0.003490658503988666988 ) ;
#39574=AXIS2_PLACEMENT_3D ( 'NONE', #17337, #65806, #57292 ) ;
#39575=CARTESIAN_POINT ( 'NONE',  ( 11.44999999999990692, 2.500000000000000000, -6.841600689897078702 ) ) ;
#39576=ORIENTED_EDGE ( 'NONE', *, *, #9483, .T. ) ;
#39578=EDGE_CURVE ( 'NONE', #30658, #39552, #100793, .T. ) ;
#39579=EDGE_LOOP ( 'NONE', ( #110721, #95209 ) ) ;
#39580=DIRECTION ( 'NONE',  ( 0.000000000000000000, -0.9999939076577903929, 0.003490651415223739937 ) ) ;
#39581=FACE_OUTER_BOUND ( 'NONE', #40481, .T. ) ;
#39582=EDGE_CURVE ( 'NONE', #124473, #36694, #126911, .T. ) ;
#39583=CIRCLE ( 'NONE', #125233, 0.1000000000000002554 ) ;
#39584=AXIS2_PLACEMENT_3D ( 'NONE', #71022, #39011, #70369 ) ;
#39585=DIRECTION ( 'NONE',  ( 0.000000000000000000, 0.000000000000000000, -1.000000000000000000 ) ) ;
#39586=DIRECTION ( 'NONE',  ( -0.000000000000000000, -1.000000000000000000, -0.000000000000000000 ) ) ;
#39587=CARTESIAN_POINT ( 'NONE',  ( -15.39999999999998082, 2.500000000000000000, 0.6928203230275518099 ) ) ;
#39588=ADVANCED_FACE ( 'NONE', ( #22275 ), #64196, .T. ) ;
#39590=DIRECTION ( 'NONE',  ( -0.000000000000000000, -1.000000000000000000, -0.000000000000000000 ) ) ;
#39591=ORIENTED_EDGE ( 'NONE', *, *, #23607, .T. ) ;
#39592=ADVANCED_FACE ( 'NONE', ( #111927 ), #34989, .T. ) ;
#39593=CIRCLE ( 'NONE', #118976, 0.1000000000000000472 ) ;
#39594=AXIS2_PLACEMENT_3D ( 'NONE', #98629, #129431, #51498 ) ;
#39595=CARTESIAN_POINT ( 'NONE',  ( -3.950000000000024603, 2.500000000000000000, 1.918653347947321564 ) ) ;
#39596=EDGE_CURVE ( 'NONE', #16787, #127183, #108118, .T. ) ;
#39597=FACE_OUTER_BOUND ( 'NONE', #101679, .T. ) ;
#39598=ORIENTED_EDGE ( 'NONE', *, *, #78567, .F. ) ;
#39599=EDGE_CURVE ( 'NONE', #48770, #98786, #52353, .T. ) ;
#39600=DIRECTION ( 'NONE',  ( -0.000000000000000000, -1.000000000000000000, -0.000000000000000000 ) ) ;
#39601=ORIENTED_EDGE ( 'NONE', *, *, #20934, .T. ) ;
#39602=VERTEX_POINT ( 'NONE', #123653 ) ;
#39603=DIRECTION ( 'NONE',  ( 0.000000000000000000, 1.000000000000000000, 0.000000000000000000 ) ) ;
#39604=VERTEX_POINT ( 'NONE', #23531 ) ;
#39605=CARTESIAN_POINT ( 'NONE',  ( 7.899999999999923084, 12.50000000000000000, 0.7579135962115869374 ) ) ;
#39606=DIRECTION ( 'NONE',  ( 0.000000000000000000, 0.000000000000000000, 1.000000000000000000 ) ) ;
#39607=ORIENTED_EDGE ( 'NONE', *, *, #117683, .T. ) ;
#39608=CONICAL_SURFACE ( 'NONE', #20800, 0.09999999999999982514, 0.003490658503988666988 ) ;
#39609=LINE ( 'NONE', #69682, #38397 ) ;
#39610=AXIS2_PLACEMENT_3D ( 'NONE', #67343, #87650, #117745 ) ;
#39611=CARTESIAN_POINT ( 'NONE',  ( -8.150000000000014566, 2.500000000000000000, -6.941600689897073906 ) ) ;
#39612=EDGE_LOOP ( 'NONE', ( #75809, #40194 ) ) ;
#39613=CARTESIAN_POINT ( 'NONE',  ( -3.350000000000028511, 12.50000000000000000, 1.472243186433545459 ) ) ;
#39614=ADVANCED_FACE ( 'NONE', ( #83751 ), #120647, .T. ) ;
#39615=AXIS2_PLACEMENT_3D ( 'NONE', #65618, #76736, #85263 ) ;
#39616=ORIENTED_EDGE ( 'NONE', *, *, #67123, .F. ) ;
#39617=CIRCLE ( 'NONE', #89761, 0.06509327318403745899 ) ;
#39618=CIRCLE ( 'NONE', #64626, 0.06509327318403745899 ) ;
#39619=EDGE_LOOP ( 'NONE', ( #120088, #53349, #63646, #99835 ) ) ;
#39620=ORIENTED_EDGE ( 'NONE', *, *, #128199, .F. ) ;
#39621=PLANE ( 'NONE',  #111045 ) ;
#39622=LINE ( 'NONE', #79523, #68841 ) ;
#39623=CARTESIAN_POINT ( 'NONE',  ( -6.850000000000017408, 2.500000000000000000, -1.918653347947325782 ) ) ;
#39624=FACE_BOUND ( 'NONE', #123577, .T. ) ;
#39625=ORIENTED_EDGE ( 'NONE', *, *, #78843, .F. ) ;
#39626=AXIS2_PLACEMENT_3D ( 'NONE', #82091, #32383, #21232 ) ;
#39627=DIRECTION ( 'NONE',  ( 0.000000000000000000, 1.000000000000000000, 0.000000000000000000 ) ) ;
#39628=CARTESIAN_POINT ( 'NONE',  ( -12.09999999999999609, 2.500000000000000000, -0.6928203230275501445 ) ) ;
#39629=ORIENTED_EDGE ( 'NONE', *, *, #78075, .T. ) ;
#39630=AXIS2_PLACEMENT_3D ( 'NONE', #89293, #119384, #29725 ) ;
#39631=CARTESIAN_POINT ( 'NONE',  ( 9.349999999999919709, 12.50000000000000000, 2.511473670974873507 ) ) ;
#39632=FACE_OUTER_BOUND ( 'NONE', #84599, .T. ) ;
#39633=CIRCLE ( 'NONE', #43828, 0.1000000000000002554 ) ;
#39635=CARTESIAN_POINT ( 'NONE',  ( 11.84999999999990372, 2.500000000000000000, -6.741600689897078169 ) ) ;
#39636=DIRECTION ( 'NONE',  ( 0.000000000000000000, 0.000000000000000000, 1.000000000000000000 ) ) ;
#39637=DIRECTION ( 'NONE',  ( 0.000000000000000000, 0.000000000000000000, 1.000000000000000000 ) ) ;
#39638=LINE ( 'NONE', #68411, #112065 ) ;
#39639=CARTESIAN_POINT ( 'NONE',  ( -6.900000000000019007, 12.50000000000000000, -0.4115034346978157509 ) ) ;
#39640=ORIENTED_EDGE ( 'NONE', *, *, #100595, .T. ) ;
#39641=ORIENTED_EDGE ( 'NONE', *, *, #64325, .F. ) ;
#39643=ORIENTED_EDGE ( 'NONE', *, *, #29648, .F. ) ;
#39644=VERTEX_POINT ( 'NONE', #26126 ) ;
#39645=AXIS2_PLACEMENT_3D ( 'NONE', #78358, #48901, #88803 ) ;
#39646=FACE_OUTER_BOUND ( 'NONE', #21097, .T. ) ;
#39647=DIRECTION ( 'NONE',  ( 0.000000000000000000, 1.000000000000000000, 0.000000000000000000 ) ) ;
#39648=EDGE_LOOP ( 'NONE', ( #63622, #60124 ) ) ;
#39649=EDGE_CURVE ( 'NONE', #52738, #94125, #43295, .T. ) ;
#39650=FACE_BOUND ( 'NONE', #37489, .T. ) ;
#39651=CARTESIAN_POINT ( 'NONE',  ( 8.749999999999920064, 2.500000000000000000, -2.957883832488653830 ) ) ;
#39652=DIRECTION ( 'NONE',  ( -0.000000000000000000, 1.000000000000000000, -0.000000000000000000 ) ) ;
#39653=DIRECTION ( 'NONE',  ( 0.000000000000000000, 1.000000000000000000, 0.000000000000000000 ) ) ;
#39654=DIRECTION ( 'NONE',  ( 0.000000000000000000, 0.000000000000000000, 1.000000000000000000 ) ) ;
#39655=DIRECTION ( 'NONE',  ( -4.274815082592931898E-19, -0.9999939076577903929, -0.003490651415223739937 ) ) ;
#39656=DIRECTION ( 'NONE',  ( 0.000000000000000000, -0.000000000000000000, 1.000000000000000000 ) ) ;
#39657=VERTEX_POINT ( 'NONE', #5813 ) ;
#39658=AXIS2_PLACEMENT_3D ( 'NONE', #76705, #7299, #87795 ) ;
#39659=VERTEX_POINT ( 'NONE', #64105 ) ;
#39660=VERTEX_POINT ( 'NONE', #46389 ) ;
#39661=VERTEX_POINT ( 'NONE', #104040 ) ;
#39662=ORIENTED_EDGE ( 'NONE', *, *, #22464, .T. ) ;
#39663=CARTESIAN_POINT ( 'NONE',  ( 14.93723468728821580, 2.499999999999999556, 6.174425104148618892 ) ) ;
#39664=CARTESIAN_POINT ( 'NONE',  ( 17.49862860983166257, -2.500000000000000000, -4.081131818001380474 ) ) ;
#39665=CONICAL_SURFACE ( 'NONE', #112804, 0.09999999999999999167, 0.003490658503988666988 ) ;
#39666=VERTEX_POINT ( 'NONE', #45772 ) ;
#39667=CARTESIAN_POINT ( 'NONE',  ( 6.249999999999932498, 2.500000000000000000, -2.757883832488654097 ) ) ;
#39668=CARTESIAN_POINT ( 'NONE',  ( -0.8000000000000376810, 2.500000000000000000, -4.430127018922202176 ) ) ;
#39669=EDGE_CURVE ( 'NONE', #70557, #87886, #70466, .T. ) ;
#39670=CIRCLE ( 'NONE', #129464, 0.06509327318403745899 ) ;
#39671=DIRECTION ( 'NONE',  ( 0.000000000000000000, 1.000000000000000000, 0.000000000000000000 ) ) ;
#39672=VECTOR ( 'NONE', #50867, 1000.000000000000000 ) ;
#39673=DIRECTION ( 'NONE',  ( -0.000000000000000000, 1.000000000000000000, -0.000000000000000000 ) ) ;
#39674=CARTESIAN_POINT ( 'NONE',  ( 12.49999999999993960, 2.500000000000000000, 4.330127018922196314 ) ) ;
#39675=LINE ( 'NONE', #32437, #78178 ) ;
#39676=AXIS2_PLACEMENT_3D ( 'NONE', #34981, #64410, #65035 ) ;
#39678=EDGE_LOOP ( 'NONE', ( #117294, #73739 ) ) ;
#39679=DIRECTION ( 'NONE',  ( 0.000000000000000000, -0.9999939076577903929, 0.003490651415223739937 ) ) ;
#39680=EDGE_CURVE ( 'NONE', #57147, #14174, #7762, .T. ) ;
#39682=AXIS2_PLACEMENT_3D ( 'NONE', #23003, #32834, #41370 ) ;
#39683=ORIENTED_EDGE ( 'NONE', *, *, #4734, .T. ) ;
#39684=ORIENTED_EDGE ( 'NONE', *, *, #23770, .F. ) ;
#39685=CARTESIAN_POINT ( 'NONE',  ( 1.249999999999986899, 2.500000000000000000, 6.495190528383297135 ) ) ;
#39686=EDGE_CURVE ( 'NONE', #75669, #65538, #112430, .T. ) ;
#39687=DIRECTION ( 'NONE',  ( 0.000000000000000000, 1.000000000000000000, 0.000000000000000000 ) ) ;
#39688=CARTESIAN_POINT ( 'NONE',  ( -2.700000000000030376, 2.500000000000000000, 3.983716857408420964 ) ) ;
#39689=EDGE_CURVE ( 'NONE', #92601, #109495, #116519, .T. ) ;
#39690=EDGE_CURVE ( 'NONE', #128991, #11848, #26656, .T. ) ;
#39692=ORIENTED_EDGE ( 'NONE', *, *, #95409, .F. ) ;
#39693=VERTEX_POINT ( 'NONE', #76515 ) ;
#39694=FACE_OUTER_BOUND ( 'NONE', #11496, .T. ) ;
#39695=DIRECTION ( 'NONE',  ( -0.000000000000000000, 1.000000000000000000, -0.000000000000000000 ) ) ;
#39696=EDGE_CURVE ( 'NONE', #65503, #129420, #72713, .T. ) ;
#39697=CARTESIAN_POINT ( 'NONE',  ( -9.400000000000007461, 12.50000000000000000, -0.3464101615137783474 ) ) ;
#39698=EDGE_CURVE ( 'NONE', #50747, #86566, #114466, .T. ) ;
#39699=CARTESIAN_POINT ( 'NONE',  ( 3.149999999999944400, 12.50000000000000000, 2.511473670974873507 ) ) ;
#39700=ORIENTED_EDGE ( 'NONE', *, *, #47219, .F. ) ;
#39701=ADVANCED_FACE ( 'NONE', ( #124322 ), #26766, .T. ) ;
#39702=CARTESIAN_POINT ( 'NONE',  ( -2.100000000000033396, 2.500000000000000000, -5.022947341949754119 ) ) ;
#39703=ADVANCED_FACE ( 'NONE', ( #104661 ), #24192, .T. ) ;
#39704=ORIENTED_EDGE ( 'NONE', *, *, #14959, .F. ) ;
#39705=CARTESIAN_POINT ( 'NONE',  ( -11.44999999999999929, 2.500000000000000000, -1.918653347947322230 ) ) ;
#39706=EDGE_CURVE ( 'NONE', #89734, #16131, #65387, .T. ) ;
#39707=AXIS2_PLACEMENT_3D ( 'NONE', #61137, #30412, #9460 ) ;
#39708=ADVANCED_FACE ( 'NONE', ( #85027 ), #89436, .T. ) ;
#39709=ORIENTED_EDGE ( 'NONE', *, *, #70683, .T. ) ;
#39710=DIRECTION ( 'NONE',  ( 0.000000000000000000, 0.000000000000000000, 1.000000000000000000 ) ) ;
#39711=CARTESIAN_POINT ( 'NONE',  ( 87.50000000000001421, -3.975344334345451980, 6.360552532166690476 ) ) ;
#39712=CARTESIAN_POINT ( 'NONE',  ( -1.050000000000038680, 2.500000000000000000, 2.511473670974873507 ) ) ;
#39713=PLANE ( 'NONE',  #104428 ) ;
#39714=EDGE_CURVE ( 'NONE', #42111, #56218, #33019, .T. ) ;
#39715=ORIENTED_EDGE ( 'NONE', *, *, #52228, .T. ) ;
#39716=CIRCLE ( 'NONE', #98156, 0.06509327318403745899 ) ;
#39717=VECTOR ( 'NONE', #104841, 1000.000000000000000 ) ;
#39718=DIRECTION ( 'NONE',  ( 0.000000000000000000, 0.000000000000000000, -1.000000000000000000 ) ) ;
#39719=ORIENTED_EDGE ( 'NONE', *, *, #72002, .F. ) ;
#39721=LINE ( 'NONE', #48882, #54106 ) ;
#39722=FACE_OUTER_BOUND ( 'NONE', #60813, .T. ) ;
#39723=CARTESIAN_POINT ( 'NONE',  ( 6.899999999999926636, 2.500000000000000000, 0.4464101615137736623 ) ) ;
#39725=CARTESIAN_POINT ( 'NONE',  ( -14.14999999999998614, 2.500000000000000000, 2.065063509461101621 ) ) ;
#39726=FACE_OUTER_BOUND ( 'NONE', #77737, .T. ) ;
#39727=AXIS2_PLACEMENT_3D ( 'NONE', #47293, #66273, #15877 ) ;
#39728=AXIS2_PLACEMENT_3D ( 'NONE', #112030, #40734, #100900 ) ;
#39729=DIRECTION ( 'NONE',  ( 0.000000000000000000, 1.000000000000000000, 0.000000000000000000 ) ) ;
#39730=DIRECTION ( 'NONE',  ( 0.000000000000000000, 0.000000000000000000, -1.000000000000000000 ) ) ;
#39731=DIRECTION ( 'NONE',  ( -4.274815082592931898E-19, -0.9999939076577903929, -0.003490651415223739937 ) ) ;
#39732=VECTOR ( 'NONE', #53737, 1000.000000000000000 ) ;
#39733=ORIENTED_EDGE ( 'NONE', *, *, #37404, .T. ) ;
#39734=PLANE ( 'NONE',  #17018 ) ;
#39735=CARTESIAN_POINT ( 'NONE',  ( 9.999999999999912959, 12.50000000000000000, -5.088040615133791356 ) ) ;
#39736=DIRECTION ( 'NONE',  ( 0.000000000000000000, 1.000000000000000000, 0.000000000000000000 ) ) ;
#39737=CARTESIAN_POINT ( 'NONE',  ( 3.749999999999940492, 12.50000000000000000, 2.922977105672686982 ) ) ;
#39738=DIRECTION ( 'NONE',  ( 0.000000000000000000, 0.000000000000000000, -1.000000000000000000 ) ) ;
#39739=ORIENTED_EDGE ( 'NONE', *, *, #20870, .F. ) ;
#39740=FACE_OUTER_BOUND ( 'NONE', #82870, .T. ) ;
#39741=EDGE_CURVE ( 'NONE', #70146, #128034, #99813, .T. ) ;
#39743=LINE ( 'NONE', #33755, #43012 ) ;
#39744=PLANE ( 'NONE',  #19693 ) ;
#39745=VERTEX_POINT ( 'NONE', #117693 ) ;
#39746=ORIENTED_EDGE ( 'NONE', *, *, #50400, .F. ) ;
#39748=DIRECTION ( 'NONE',  ( 0.000000000000000000, 0.000000000000000000, 1.000000000000000000 ) ) ;
#39749=ORIENTED_EDGE ( 'NONE', *, *, #6828, .T. ) ;
#39750=ORIENTED_EDGE ( 'NONE', *, *, #95508, .F. ) ;
#39751=ORIENTED_EDGE ( 'NONE', *, *, #17151, .F. ) ;
#39752=PLANE ( 'NONE',  #69702 ) ;
#39753=AXIS2_PLACEMENT_3D ( 'NONE', #78480, #118372, #28722 ) ;
#39754=DIRECTION ( 'NONE',  ( 0.000000000000000000, 0.000000000000000000, -1.000000000000000000 ) ) ;
#39755=CARTESIAN_POINT ( 'NONE',  ( 2.699999999999946443, 2.500000000000000000, -3.983716857408426293 ) ) ;
#39756=PLANE ( 'NONE',  #85527 ) ;
#39757=ORIENTED_EDGE ( 'NONE', *, *, #110402, .T. ) ;
#39758=AXIS2_PLACEMENT_3D ( 'NONE', #48094, #55961, #87348 ) ;
#39759=AXIS2_PLACEMENT_3D ( 'NONE', #26561, #86094, #66471 ) ;
#39760=DIRECTION ( 'NONE',  ( 0.000000000000000000, -0.000000000000000000, 1.000000000000000000 ) ) ;
#39761=EDGE_LOOP ( 'NONE', ( #104355, #94472 ) ) ;
#39762=CARTESIAN_POINT ( 'NONE',  ( -12.69999999999999218, 12.50000000000000000, 4.741630453620009789 ) ) ;
#39763=CARTESIAN_POINT ( 'NONE',  ( 19.61395058415635617, 2.556813634648583022, 4.305699210822707457 ) ) ;
#39764=DIRECTION ( 'NONE',  ( 0.000000000000000000, 1.000000000000000000, 0.000000000000000000 ) ) ;
#39765=FACE_OUTER_BOUND ( 'NONE', #24207, .T. ) ;
#39766=EDGE_LOOP ( 'NONE', ( #80423, #28686, #119198, #121937 ) ) ;
#39767=CIRCLE ( 'NONE', #123365, 0.1000000000000002554 ) ;
#39768=ORIENTED_EDGE ( 'NONE', *, *, #102197, .F. ) ;
#39769=EDGE_LOOP ( 'NONE', ( #51660, #120661, #11229, #3665 ) ) ;
#39770=VERTEX_POINT ( 'NONE', #109838 ) ;
#39771=VERTEX_POINT ( 'NONE', #47703 ) ;
#39772=CARTESIAN_POINT ( 'NONE',  ( -7.499999999999980460, 2.500000000000000000, -0.1000000000000022815 ) ) ;
#39773=DIRECTION ( 'NONE',  ( 0.000000000000000000, 0.000000000000000000, -1.000000000000000000 ) ) ;
#39774=DIRECTION ( 'NONE',  ( 0.000000000000000000, 0.000000000000000000, -1.000000000000000000 ) ) ;
#39775=FACE_BOUND ( 'NONE', #6113, .T. ) ;
#39776=DIRECTION ( 'NONE',  ( 0.000000000000000000, 0.000000000000000000, 1.000000000000000000 ) ) ;
#39778=CARTESIAN_POINT ( 'NONE',  ( 9.599999999999917932, 2.500000000000000000, -2.276824562219559311E-15 ) ) ;
#39779=CARTESIAN_POINT ( 'NONE',  ( -13.94999999999998863, 2.500000000000000000, -1.718653347947323828 ) ) ;
#39780=FACE_OUTER_BOUND ( 'NONE', #58970, .T. ) ;
#39781=CARTESIAN_POINT ( 'NONE',  ( 15.59999999999988951, 12.50000000000000000, -0.3464101615137783474 ) ) ;
#39782=FACE_OUTER_BOUND ( 'NONE', #64294, .T. ) ;
#39783=AXIS2_PLACEMENT_3D ( 'NONE', #88260, #28080, #47725 ) ;
#39784=AXIS2_PLACEMENT_3D ( 'NONE', #38868, #19847, #8073 ) ;
#39785=PLANE ( 'NONE',  #55675 ) ;
#39786=VERTEX_POINT ( 'NONE', #38546 ) ;
#39787=ORIENTED_EDGE ( 'NONE', *, *, #120891, .T. ) ;
#39788=VERTEX_POINT ( 'NONE', #87605 ) ;
#39789=VERTEX_POINT ( 'NONE', #18865 ) ;
#39790=EDGE_CURVE ( 'NONE', #24400, #54589, #62261, .T. ) ;
#39791=DIRECTION ( 'NONE',  ( 0.000000000000000000, 0.000000000000000000, -1.000000000000000000 ) ) ;
#39792=DIRECTION ( 'NONE',  ( 0.000000000000000000, 0.000000000000000000, 1.000000000000000000 ) ) ;
#39793=EDGE_CURVE ( 'NONE', #56486, #83051, #22552, .T. ) ;
#39794=FACE_BOUND ( 'NONE', #3047, .T. ) ;
#39795=AXIS2_PLACEMENT_3D ( 'NONE', #121662, #61482, #90923 ) ;
#39796=CARTESIAN_POINT ( 'NONE',  ( -0.4000000000000392131, 2.500000000000000000, -4.430127018922202176 ) ) ;
#39797=ORIENTED_EDGE ( 'NONE', *, *, #98643, .T. ) ;
#39798=DIRECTION ( 'NONE',  ( 0.000000000000000000, 0.000000000000000000, 1.000000000000000000 ) ) ;
#39799=FACE_OUTER_BOUND ( 'NONE', #76247, .T. ) ;
#39800=EDGE_CURVE ( 'NONE', #90204, #28068, #85229, .T. ) ;
#39801=DIRECTION ( 'NONE',  ( 0.000000000000000000, 0.000000000000000000, -1.000000000000000000 ) ) ;
#39802=DIRECTION ( 'NONE',  ( 0.000000000000000000, 0.000000000000000000, 1.000000000000000000 ) ) ;
#39803=CIRCLE ( 'NONE', #125455, 0.06509327318403745899 ) ;
#39804=VERTEX_POINT ( 'NONE', #109171 ) ;
#39805=DIRECTION ( 'NONE',  ( 0.000000000000000000, -0.000000000000000000, 1.000000000000000000 ) ) ;
#39806=CIRCLE ( 'NONE', #54443, 0.1000000000000002554 ) ;
#39807=AXIS2_PLACEMENT_3D ( 'NONE', #116995, #19455, #119579 ) ;
#39808=VERTEX_POINT ( 'NONE', #19512 ) ;
#39809=VERTEX_POINT ( 'NONE', #59476 ) ;
#39810=CARTESIAN_POINT ( 'NONE',  ( -12.49999999999999289, 2.500000000000000000, -0.5928203230275499447 ) ) ;
#39811=DIRECTION ( 'NONE',  ( 0.000000000000000000, 1.000000000000000000, 0.000000000000000000 ) ) ;
#39812=ORIENTED_EDGE ( 'NONE', *, *, #49299, .F. ) ;
#39813=AXIS2_PLACEMENT_3D ( 'NONE', #20905, #109280, #30752 ) ;
#39814=DIRECTION ( 'NONE',  ( -4.274815082592931898E-19, -0.9999939076577903929, -0.003490651415223739937 ) ) ;
#39815=CARTESIAN_POINT ( 'NONE',  ( 2.099999999999950351, 2.500000000000000000, -0.5928203230275541635 ) ) ;
#39816=EDGE_CURVE ( 'NONE', #31177, #127925, #95704, .T. ) ;
#39817=ORIENTED_EDGE ( 'NONE', *, *, #68482, .T. ) ;
#39818=DIRECTION ( 'NONE',  ( 0.000000000000000000, 1.000000000000000000, 0.000000000000000000 ) ) ;
#39819=CONICAL_SURFACE ( 'NONE', #4177, 0.1000000000000002554, 0.003490658503988666988 ) ;
#39820=EDGE_LOOP ( 'NONE', ( #119447, #28285 ) ) ;
#39821=DIRECTION ( 'NONE',  ( -0.000000000000000000, -1.000000000000000000, -0.000000000000000000 ) ) ;
#39822=ORIENTED_EDGE ( 'NONE', *, *, #75437, .F. ) ;
#39823=FACE_BOUND ( 'NONE', #4996, .T. ) ;
#39824=EDGE_CURVE ( 'NONE', #37787, #97225, #79730, .T. ) ;
#39825=ORIENTED_EDGE ( 'NONE', *, *, #100963, .T. ) ;
#39826=DIRECTION ( 'NONE',  ( -0.000000000000000000, 1.000000000000000000, -0.000000000000000000 ) ) ;
#39827=ORIENTED_EDGE ( 'NONE', *, *, #50173, .F. ) ;
#39828=DIRECTION ( 'NONE',  ( 0.000000000000000000, 0.000000000000000000, 1.000000000000000000 ) ) ;
#39829=CARTESIAN_POINT ( 'NONE',  ( -7.300000000000018474, 2.500000000000000000, 0.3464101615137735735 ) ) ;
#39830=EDGE_CURVE ( 'NONE', #37733, #120555, #83093, .T. ) ;
#39831=CARTESIAN_POINT ( 'NONE',  ( -4.150000000000024336, 2.500000000000000000, 2.165063509461097713 ) ) ;
#39833=EDGE_CURVE ( 'NONE', #77015, #12520, #76829, .T. ) ;
#39834=ADVANCED_FACE ( 'NONE', ( #101950 ), #74773, .T. ) ;
#39835=CARTESIAN_POINT ( 'NONE',  ( -8.950000000000009948, 12.50000000000000000, 2.446380397790835826 ) ) ;
#39836=EDGE_CURVE ( 'NONE', #109336, #34349, #74268, .T. ) ;
#39837=ORIENTED_EDGE ( 'NONE', *, *, #81404, .F. ) ;
#39838=ORIENTED_EDGE ( 'NONE', *, *, #33077, .F. ) ;
#39839=ORIENTED_EDGE ( 'NONE', *, *, #12136, .T. ) ;
#39840=DIRECTION ( 'NONE',  ( 0.000000000000000000, 1.000000000000000000, 0.000000000000000000 ) ) ;
#39841=DIRECTION ( 'NONE',  ( -0.000000000000000000, 1.000000000000000000, -0.000000000000000000 ) ) ;
#39842=ADVANCED_FACE ( 'NONE', ( #92114 ), #2438, .T. ) ;
#39843=CIRCLE ( 'NONE', #117150, 0.1000000000000002554 ) ;
#39844=DIRECTION ( 'NONE',  ( 0.000000000000000000, 0.000000000000000000, -1.000000000000000000 ) ) ;
#39845=ORIENTED_EDGE ( 'NONE', *, *, #19450, .T. ) ;
#39847=ORIENTED_EDGE ( 'NONE', *, *, #62616, .T. ) ;
#39848=VECTOR ( 'NONE', #86823, 1000.000000000000000 ) ;
#39849=EDGE_CURVE ( 'NONE', #107424, #2395, #11630, .T. ) ;
#39850=CARTESIAN_POINT ( 'NONE',  ( -6.450000000000019718, 2.500000000000000000, -1.818653347947326138 ) ) ;
#39851=EDGE_LOOP ( 'NONE', ( #76739, #28838, #124041, #105818 ) ) ;
#39852=DIRECTION ( 'NONE',  ( 0.000000000000000000, 1.000000000000000000, 0.000000000000000000 ) ) ;
#39854=ADVANCED_FACE ( 'NONE', ( #51572 ), #129176, .T. ) ;
#39855=DIRECTION ( 'NONE',  ( -0.000000000000000000, -1.000000000000000000, -0.000000000000000000 ) ) ;
#39856=DIRECTION ( 'NONE',  ( 0.000000000000000000, 0.000000000000000000, 1.000000000000000000 ) ) ;
#39857=DIRECTION ( 'NONE',  ( 0.000000000000000000, 0.000000000000000000, 1.000000000000000000 ) ) ;
#39858=FACE_OUTER_BOUND ( 'NONE', #584, .T. ) ;
#39859=CARTESIAN_POINT ( 'NONE',  ( -6.450000000000014388, 2.500000000000000000, 1.818653347947321475 ) ) ;
#39860=EDGE_CURVE ( 'NONE', #20844, #104463, #28805, .T. ) ;
#39861=CARTESIAN_POINT ( 'NONE',  ( -9.350000000000006750, 2.500000000000000000, -2.411473670974877859 ) ) ;
#39862=EDGE_CURVE ( 'NONE', #116681, #15958, #101958, .T. ) ;
#39863=ORIENTED_EDGE ( 'NONE', *, *, #42955, .F. ) ;
#39864=ORIENTED_EDGE ( 'NONE', *, *, #69851, .T. ) ;
#39865=DIRECTION ( 'NONE',  ( 0.000000000000000000, 0.000000000000000000, 1.000000000000000000 ) ) ;
#39866=ORIENTED_EDGE ( 'NONE', *, *, #19684, .T. ) ;
#39867=VERTEX_POINT ( 'NONE', #111772 ) ;
#39868=CARTESIAN_POINT ( 'NONE',  ( 1.649999999999951950, 2.500000000000000000, -7.288010851410854585 ) ) ;
#39869=LINE ( 'NONE', #16937, #36473 ) ;
#39870=DIRECTION ( 'NONE',  ( 0.000000000000000000, 0.000000000000000000, 1.000000000000000000 ) ) ;
#39871=DIRECTION ( 'NONE',  ( 0.000000000000000000, -0.9999939076577903929, 0.003490651415223739937 ) ) ;
#39872=CARTESIAN_POINT ( 'NONE',  ( 3.749999999999975131, 2.500000000000000000, 6.595190528383296780 ) ) ;
#39873=DIRECTION ( 'NONE',  ( 0.000000000000000000, 1.000000000000000000, 0.000000000000000000 ) ) ;
#39874=CARTESIAN_POINT ( 'NONE',  ( 13.29999999999989946, 12.50000000000000000, -0.06509327318403980434 ) ) ;
#39875=DIRECTION ( 'NONE',  ( -0.000000000000000000, -1.000000000000000000, -0.000000000000000000 ) ) ;
#39876=CIRCLE ( 'NONE', #100488, 0.06509327318403745899 ) ;
#39877=AXIS2_PLACEMENT_3D ( 'NONE', #13576, #54789, #24705 ) ;
#39878=EDGE_LOOP ( 'NONE', ( #123631, #82295 ) ) ;
#39879=ORIENTED_EDGE ( 'NONE', *, *, #20183, .T. ) ;
#39880=ORIENTED_EDGE ( 'NONE', *, *, #1544, .T. ) ;
#39881=ORIENTED_EDGE ( 'NONE', *, *, #119582, .F. ) ;
#39882=DIRECTION ( 'NONE',  ( -0.000000000000000000, -1.000000000000000000, -0.000000000000000000 ) ) ;
#39883=CARTESIAN_POINT ( 'NONE',  ( -11.84999999999999609, 2.500000000000000000, 6.741600689897071952 ) ) ;
#39884=CONICAL_SURFACE ( 'NONE', #113019, 0.1000000000000002554, 0.003490658503988666988 ) ;
#39885=VERTEX_POINT ( 'NONE', #65065 ) ;
#39886=DIRECTION ( 'NONE',  ( -0.000000000000000000, -1.000000000000000000, -0.000000000000000000 ) ) ;
#39887=EDGE_CURVE ( 'NONE', #120491, #47940, #91486, .T. ) ;
#39888=DIRECTION ( 'NONE',  ( 0.000000000000000000, 0.000000000000000000, -1.000000000000000000 ) ) ;
#39889=ADVANCED_FACE ( 'NONE', ( #30646 ), #10959, .T. ) ;
#39890=LINE ( 'NONE', #71254, #65771 ) ;
#39892=ORIENTED_EDGE ( 'NONE', *, *, #7695, .T. ) ;
#39893=( BOUNDED_SURFACE ( )  B_SPLINE_SURFACE ( 3, 2, ( 
 ( #98865, #9200, #49150 ),
 ( #89058, #129008, #26913 ),
 ( #28203, #69400, #68113 ),
 ( #47854, #39337, #109334 ) ),
 .UNSPECIFIED., .F., .F., .F. ) 
 B_SPLINE_SURFACE_WITH_KNOTS ( ( 4, 4 ),
 ( 3, 3 ),
 ( 0.000000000000000000, 0.002140783067917607571 ),
 ( 0.000000000000000000, 1.000000000000000000 ),
 .UNSPECIFIED. ) 
 GEOMETRIC_REPRESENTATION_ITEM ( )  RATIONAL_B_SPLINE_SURFACE ( (
 ( 1.000000000000000000, 0.7071067811865471286, 1.000000000000000000),
 ( 1.000000000000000000, 0.7083221562484207645, 1.000000000000000000),
 ( 1.000000000000000000, 0.7095583416414845690, 1.000000000000000000),
 ( 1.000000000000000000, 0.7108129113927459386, 1.000000000000000000) ) ) 
 REPRESENTATION_ITEM ( '' )  SURFACE ( )  );
#39894=DIRECTION ( 'NONE',  ( 0.000000000000000000, 0.000000000000000000, -1.000000000000000000 ) ) ;
#39895=DIRECTION ( 'NONE',  ( 0.000000000000000000, 1.000000000000000000, 0.000000000000000000 ) ) ;
#39896=AXIS2_PLACEMENT_3D ( 'NONE', #121657, #113128, #111181 ) ;
#39897=ORIENTED_EDGE ( 'NONE', *, *, #21998, .T. ) ;
#39898=AXIS2_PLACEMENT_3D ( 'NONE', #442, #60056, #71791 ) ;
#39899=EDGE_LOOP ( 'NONE', ( #46816, #60776, #7193, #98671 ) ) ;
#39900=EDGE_LOOP ( 'NONE', ( #45653, #115537 ) ) ;
#39901=VERTEX_POINT ( 'NONE', #101313 ) ;
#39902=DIRECTION ( 'NONE',  ( 0.000000000000000000, -0.000000000000000000, 1.000000000000000000 ) ) ;
#39903=AXIS2_PLACEMENT_3D ( 'NONE', #24781, #114431, #84975 ) ;
#39904=CARTESIAN_POINT ( 'NONE',  ( 8.749999999999957367, 2.500000000000000000, -6.495190528383302464 ) ) ;
#39905=CARTESIAN_POINT ( 'NONE',  ( -14.99999999999994671, 12.50000000000000000, 0.000000000000000000 ) ) ;
#39906=AXIS2_PLACEMENT_3D ( 'NONE', #95307, #6254, #116219 ) ;
#39907=ORIENTED_EDGE ( 'NONE', *, *, #25311, .F. ) ;
#39908=DIRECTION ( 'NONE',  ( 0.000000000000000000, 0.000000000000000000, 1.000000000000000000 ) ) ;
#39909=CARTESIAN_POINT ( 'NONE',  ( 20.37757664703730853, -0.6627606010239102119, -4.188167776336774395 ) ) ;
#39910=CARTESIAN_POINT ( 'NONE',  ( -1.650000000000034772, 2.500000000000000000, 6.395190528383296602 ) ) ;
#39911=DIRECTION ( 'NONE',  ( -0.000000000000000000, 1.000000000000000000, -0.000000000000000000 ) ) ;
#39912=ORIENTED_EDGE ( 'NONE', *, *, #100947, .F. ) ;
#39913=PLANE ( 'NONE',  #29098 ) ;
#39914=ORIENTED_EDGE ( 'NONE', *, *, #104676, .T. ) ;
#39915=VERTEX_POINT ( 'NONE', #84723 ) ;
#39916=CARTESIAN_POINT ( 'NONE',  ( 13.34999999999990017, 12.50000000000000000, 2.165063509461097713 ) ) ;
#39917=CARTESIAN_POINT ( 'NONE',  ( 7.099999999999927702, 2.500000000000000000, -3.637306695894650055 ) ) ;
#39918=FACE_BOUND ( 'NONE', #95628, .T. ) ;
#39919=CARTESIAN_POINT ( 'NONE',  ( 7.299999999999927880, 12.50000000000000000, 3.983716857408420964 ) ) ;
#39920=CARTESIAN_POINT ( 'NONE',  ( 1.849999999999949685, 2.500000000000000000, 1.918653347947321564 ) ) ;
#39921=DIRECTION ( 'NONE',  ( 0.000000000000000000, 0.000000000000000000, 1.000000000000000000 ) ) ;
#39922=EDGE_CURVE ( 'NONE', #120005, #117161, #14677, .T. ) ;
#39923=CIRCLE ( 'NONE', #46163, 0.06509327318403741736 ) ;
#39924=CONICAL_SURFACE ( 'NONE', #117245, 0.09999999999999999167, 0.003490658503988666988 ) ;
#39925=LINE ( 'NONE', #99489, #27550 ) ;
#39926=AXIS2_PLACEMENT_3D ( 'NONE', #89413, #37738, #48195 ) ;
#39927=DIRECTION ( 'NONE',  ( 0.000000000000000000, 1.000000000000000000, 0.000000000000000000 ) ) ;
#39928=CARTESIAN_POINT ( 'NONE',  ( 8.099999999999923261, 2.500000000000000000, 4.083716857408420609 ) ) ;
#39929=ORIENTED_EDGE ( 'NONE', *, *, #118219, .T. ) ;
#39930=EDGE_CURVE ( 'NONE', #37231, #46960, #127002, .T. ) ;
#39931=DIRECTION ( 'NONE',  ( 0.000000000000000000, -0.000000000000000000, 1.000000000000000000 ) ) ;
#39932=LINE ( 'NONE', #100136, #68383 ) ;
#39933=ORIENTED_EDGE ( 'NONE', *, *, #17479, .F. ) ;
#39934=ORIENTED_EDGE ( 'NONE', *, *, #44062, .T. ) ;
#39935=EDGE_CURVE ( 'NONE', #106998, #108508, #104012, .T. ) ;
#39936=CARTESIAN_POINT ( 'NONE',  ( 11.84999999999990727, 12.50000000000000000, -1.818653347947326138 ) ) ;
#39938=ADVANCED_FACE ( 'NONE', ( #1166 ), #74914, .T. ) ;
#39939=FACE_BOUND ( 'NONE', #5590, .T. ) ;
#39940=CARTESIAN_POINT ( 'NONE',  ( -10.40000000000000213, 12.50000000000000000, 3.572213422710607489 ) ) ;
#39941=DIRECTION ( 'NONE',  ( 0.000000000000000000, 0.000000000000000000, 1.000000000000000000 ) ) ;
#39942=ORIENTED_EDGE ( 'NONE', *, *, #64943, .T. ) ;
#39943=CARTESIAN_POINT ( 'NONE',  ( -1.700000000000035261, 12.50000000000000000, 4.330127018922196314 ) ) ;
#39944=EDGE_CURVE ( 'NONE', #113749, #64996, #7851, .T. ) ;
#39945=CARTESIAN_POINT ( 'NONE',  ( -6.450000000000017941, 12.50000000000000000, -6.841600689897077814 ) ) ;
#39946=EDGE_LOOP ( 'NONE', ( #5324, #15850, #13325, #9185 ) ) ;
#39947=LINE ( 'NONE', #69385, #5041 ) ;
#39948=DIRECTION ( 'NONE',  ( 0.000000000000000000, 0.000000000000000000, -1.000000000000000000 ) ) ;
#39949=CIRCLE ( 'NONE', #54586, 0.09999999999999982514 ) ;
#39951=DIRECTION ( 'NONE',  ( 0.000000000000000000, 1.000000000000000000, 0.000000000000000000 ) ) ;
#39952=VECTOR ( 'NONE', #58860, 1000.000000000000000 ) ;
#39953=CIRCLE ( 'NONE', #77582, 0.1000000000000000472 ) ;
#39954=EDGE_LOOP ( 'NONE', ( #90915, #97414 ) ) ;
#39955=CARTESIAN_POINT ( 'NONE',  ( -2.500000000000031086, 12.50000000000000000, 3.572213422710607489 ) ) ;
#39956=DIRECTION ( 'NONE',  ( -0.000000000000000000, 1.000000000000000000, -0.000000000000000000 ) ) ;
#39957=DIRECTION ( 'NONE',  ( 0.000000000000000000, 1.000000000000000000, 0.000000000000000000 ) ) ;
#39958=DIRECTION ( 'NONE',  ( 0.000000000000000000, 1.000000000000000000, 0.000000000000000000 ) ) ;
#39959=EDGE_LOOP ( 'NONE', ( #24361, #51981 ) ) ;
#39960=VERTEX_POINT ( 'NONE', #5503 ) ;
#39961=DIRECTION ( 'NONE',  ( 0.000000000000000000, 1.000000000000000000, 0.000000000000000000 ) ) ;
#39962=CIRCLE ( 'NONE', #113109, 0.06509327318403741736 ) ;
#39963=VERTEX_POINT ( 'NONE', #81022 ) ;
#39964=FACE_OUTER_BOUND ( 'NONE', #79875, .T. ) ;
#39965=AXIS2_PLACEMENT_3D ( 'NONE', #2632, #22318, #12463 ) ;
#39966=CARTESIAN_POINT ( 'NONE',  ( 87.50000000000000000, -7.032605354647524010, -2.693424153406288823 ) ) ;
#39967=EDGE_CURVE ( 'NONE', #100871, #79060, #51791, .T. ) ;
#39968=LINE ( 'NONE', #100173, #50796 ) ;
#39969=ORIENTED_EDGE ( 'NONE', *, *, #88293, .F. ) ;
#39970=DIRECTION ( 'NONE',  ( 0.000000000000000000, 0.000000000000000000, -1.000000000000000000 ) ) ;
#39971=DIRECTION ( 'NONE',  ( -0.000000000000000000, -1.000000000000000000, -0.000000000000000000 ) ) ;
#39972=DIRECTION ( 'NONE',  ( -4.274815082592931898E-19, -0.9999939076577903929, -0.003490651415223739937 ) ) ;
#39973=CARTESIAN_POINT ( 'NONE',  ( 4.149999999999941735, 2.500000000000000000, -2.857883832488653741 ) ) ;
#39974=DIRECTION ( 'NONE',  ( 0.000000000000000000, 1.000000000000000000, 0.000000000000000000 ) ) ;
#39975=EDGE_CURVE ( 'NONE', #121075, #70528, #68499, .T. ) ;
#39976=CARTESIAN_POINT ( 'NONE',  ( 9.349999999999916156, 2.500000000000000000, 6.941600689897073018 ) ) ;
#39977=EDGE_CURVE ( 'NONE', #75731, #91809, #125300, .T. ) ;
#39978=AXIS2_PLACEMENT_3D ( 'NONE', #68535, #117608, #27309 ) ;
#39979=ORIENTED_EDGE ( 'NONE', *, *, #70825, .T. ) ;
#39980=VECTOR ( 'NONE', #19956, 1000.000000000000000 ) ;
#39981=ORIENTED_EDGE ( 'NONE', *, *, #112931, .T. ) ;
#39982=CARTESIAN_POINT ( 'NONE',  ( 2.099999999999949463, 2.500000000000000000, -3.637306695894650055 ) ) ;
#39983=ORIENTED_EDGE ( 'NONE', *, *, #78683, .T. ) ;
#39985=ADVANCED_FACE ( 'NONE', ( #105664 ), #17244, .T. ) ;
#39986=VERTEX_POINT ( 'NONE', #85991 ) ;
#39987=ORIENTED_EDGE ( 'NONE', *, *, #21025, .F. ) ;
#39989=ORIENTED_EDGE ( 'NONE', *, *, #128504, .F. ) ;
#39990=EDGE_CURVE ( 'NONE', #47267, #77184, #24688, .T. ) ;
#39991=FACE_OUTER_BOUND ( 'NONE', #75164, .T. ) ;
#39992=VECTOR ( 'NONE', #44912, 1000.000000000000000 ) ;
#39993=EDGE_CURVE ( 'NONE', #126433, #115678, #70650, .T. ) ;
#39994=DIRECTION ( 'NONE',  ( 0.000000000000000000, 0.000000000000000000, 1.000000000000000000 ) ) ;
#39995=CARTESIAN_POINT ( 'NONE',  ( -11.25000000000000178, 12.50000000000000000, -5.802370205355746435 ) ) ;
#39996=ADVANCED_FACE ( 'NONE', ( #17910 ), #76909, .T. ) ;
#39997=DIRECTION ( 'NONE',  ( -4.274815082592931898E-19, -0.9999939076577903929, -0.003490651415223739937 ) ) ;
#39998=AXIS2_PLACEMENT_3D ( 'NONE', #104326, #27057, #84681 ) ;
#39999=AXIS2_PLACEMENT_3D ( 'NONE', #124194, #33256, #35184 ) ;
#40000=DIRECTION ( 'NONE',  ( 0.000000000000000000, 1.000000000000000000, 0.000000000000000000 ) ) ;
#40002=DIRECTION ( 'NONE',  ( 0.000000000000000000, 0.000000000000000000, 1.000000000000000000 ) ) ;
#40003=CARTESIAN_POINT ( 'NONE',  ( 13.74999999999993427, 2.500000000000000000, 2.165063509461097713 ) ) ;
#40004=DIRECTION ( 'NONE',  ( 0.000000000000000000, -0.000000000000000000, 1.000000000000000000 ) ) ;
#40005=EDGE_CURVE ( 'NONE', #15792, #77218, #97124, .T. ) ;
#40006=EDGE_LOOP ( 'NONE', ( #84142, #123286, #118928, #103056 ) ) ;
#40007=VERTEX_POINT ( 'NONE', #46743 ) ;
#40008=DIRECTION ( 'NONE',  ( 0.000000000000000000, 1.000000000000000000, 0.000000000000000000 ) ) ;
#40009=EDGE_LOOP ( 'NONE', ( #87018, #99047, #59133, #94523 ) ) ;
#40010=ORIENTED_EDGE ( 'NONE', *, *, #54603, .T. ) ;
#40011=CARTESIAN_POINT ( 'NONE',  ( 1.649999999999951061, 12.50000000000000000, -6.560283801567339701 ) ) ;
#40012=CARTESIAN_POINT ( 'NONE',  ( -5.850000000000021849, 2.500000000000000000, -2.957883832488653830 ) ) ;
#40013=LINE ( 'NONE', #60925, #67342 ) ;
#40014=DIRECTION ( 'NONE',  ( -0.000000000000000000, 1.000000000000000000, -0.000000000000000000 ) ) ;
#40015=AXIS2_PLACEMENT_3D ( 'NONE', #113235, #42596, #63512 ) ;
#40016=DIRECTION ( 'NONE',  ( 0.000000000000000000, 1.000000000000000000, 0.000000000000000000 ) ) ;
#40017=VERTEX_POINT ( 'NONE', #87293 ) ;
#40018=CIRCLE ( 'NONE', #272, 0.06509327318403745899 ) ;
#40019=AXIS2_PLACEMENT_3D ( 'NONE', #59168, #107610, #99086 ) ;
#40020=ORIENTED_EDGE ( 'NONE', *, *, #69369, .F. ) ;
#40021=DIRECTION ( 'NONE',  ( -0.000000000000000000, -1.000000000000000000, -0.000000000000000000 ) ) ;
#40022=AXIS2_PLACEMENT_3D ( 'NONE', #66119, #6520, #77235 ) ;
#40023=ORIENTED_EDGE ( 'NONE', *, *, #103814, .F. ) ;
#40024=AXIS2_PLACEMENT_3D ( 'NONE', #16759, #105155, #55427 ) ;
#40025=ORIENTED_EDGE ( 'NONE', *, *, #33624, .F. ) ;
#40026=VECTOR ( 'NONE', #87303, 1000.000000000000000 ) ;
#40027=ORIENTED_EDGE ( 'NONE', *, *, #124342, .F. ) ;
#40028=CARTESIAN_POINT ( 'NONE',  ( 3.749999999999940492, 2.500000000000000000, 2.757883832488649656 ) ) ;
#40029=DIRECTION ( 'NONE',  ( -4.274815082592931898E-19, -0.9999939076577903929, -0.003490651415223739937 ) ) ;
#40030=FACE_OUTER_BOUND ( 'NONE', #72335, .T. ) ;
#40031=EDGE_CURVE ( 'NONE', #39771, #16038, #28901, .T. ) ;
#40032=CARTESIAN_POINT ( 'NONE',  ( 0.8499999999999527933, 2.500000000000000000, 7.188010851410848723 ) ) ;
#40033=FACE_OUTER_BOUND ( 'NONE', #45212, .T. ) ;
#40034=VERTEX_POINT ( 'NONE', #47391 ) ;
#40035=DIRECTION ( 'NONE',  ( 0.000000000000000000, 1.000000000000000000, 0.000000000000000000 ) ) ;
#40036=LINE ( 'NONE', #79945, #55781 ) ;
#40037=DIRECTION ( 'NONE',  ( 0.000000000000000000, 0.000000000000000000, 1.000000000000000000 ) ) ;
#40038=DIRECTION ( 'NONE',  ( 0.000000000000000000, 0.000000000000000000, -1.000000000000000000 ) ) ;
#40039=CARTESIAN_POINT ( 'NONE',  ( 12.49999999999990052, 2.500000000000000000, 0.5928203230275495006 ) ) ;
#40040=ADVANCED_FACE ( 'NONE', ( #65725 ), #28395, .T. ) ;
#40041=VERTEX_POINT ( 'NONE', #55905 ) ;
#40042=ORIENTED_EDGE ( 'NONE', *, *, #88118, .F. ) ;
#40043=DIRECTION ( 'NONE',  ( -0.000000000000000000, -1.000000000000000000, -0.000000000000000000 ) ) ;
#40044=ORIENTED_EDGE ( 'NONE', *, *, #92673, .T. ) ;
#40045=CARTESIAN_POINT ( 'NONE',  ( 4.799999999999935874, 2.500000000000000000, 3.983716857408420964 ) ) ;
#40046=AXIS2_PLACEMENT_3D ( 'NONE', #86211, #68514, #37779 ) ;
#40047=DIRECTION ( 'NONE',  ( 0.000000000000000000, 0.000000000000000000, -1.000000000000000000 ) ) ;
#40048=CIRCLE ( 'NONE', #8622, 0.1000000000000002554 ) ;
#40049=ORIENTED_EDGE ( 'NONE', *, *, #75726, .F. ) ;
#40050=DIRECTION ( 'NONE',  ( 0.000000000000000000, -0.000000000000000000, 1.000000000000000000 ) ) ;
#40051=CARTESIAN_POINT ( 'NONE',  ( 11.04999999999990656, 12.50000000000000000, 2.446380397790835826 ) ) ;
#40052=CARTESIAN_POINT ( 'NONE',  ( -7.500000000000001776, -2.500000000000000000, -9.000000000000000000 ) ) ;
#40053=CARTESIAN_POINT ( 'NONE',  ( -5.850000000000021849, 2.500000000000000000, -7.188010851410854052 ) ) ;
#40054=AXIS2_PLACEMENT_3D ( 'NONE', #41846, #41206, #21543 ) ;
#40055=CIRCLE ( 'NONE', #52567, 0.09999999999999982514 ) ;
#40056=CARTESIAN_POINT ( 'NONE',  ( -10.85000000000000142, 2.500000000000000000, 2.065063509461097624 ) ) ;
#40057=CONICAL_SURFACE ( 'NONE', #88138, 0.1000000000000000472, 0.003490658503988666988 ) ;
#40058=EDGE_LOOP ( 'NONE', ( #38157, #125915, #45592, #7431 ) ) ;
#40059=CARTESIAN_POINT ( 'NONE',  ( 14.59999999999989484, 12.50000000000000000, -0.6277270498435166823 ) ) ;
#40060=DIRECTION ( 'NONE',  ( 0.000000000000000000, 1.000000000000000000, 0.000000000000000000 ) ) ;
#40061=CARTESIAN_POINT ( 'NONE',  ( -15.19999999999998330, 12.50000000000000000, 0.4115034346978132529 ) ) ;
#40062=AXIS2_PLACEMENT_3D ( 'NONE', #100569, #10884, #80309 ) ;
#40063=AXIS2_PLACEMENT_3D ( 'NONE', #23162, #43472, #34298 ) ;
#40064=EDGE_CURVE ( 'NONE', #117090, #13161, #56059, .T. ) ;
#40065=VERTEX_POINT ( 'NONE', #45467 ) ;
#40066=DIRECTION ( 'NONE',  ( 0.000000000000000000, 1.000000000000000000, 0.000000000000000000 ) ) ;
#40067=AXIS2_PLACEMENT_3D ( 'NONE', #18130, #128099, #37786 ) ;
#40068=ORIENTED_EDGE ( 'NONE', *, *, #112203, .T. ) ;
#40069=DIRECTION ( 'NONE',  ( 0.000000000000000000, 0.000000000000000000, 1.000000000000000000 ) ) ;
#40070=DIRECTION ( 'NONE',  ( 0.000000000000000000, -0.000000000000000000, 1.000000000000000000 ) ) ;
#40071=AXIS2_PLACEMENT_3D ( 'NONE', #99807, #98493, #29770 ) ;
#40072=PLANE ( 'NONE',  #7842 ) ;
#40073=ORIENTED_EDGE ( 'NONE', *, *, #66656, .T. ) ;
#40074=EDGE_CURVE ( 'NONE', #111424, #33882, #79077, .T. ) ;
#40075=DIRECTION ( 'NONE',  ( 0.000000000000000000, 1.000000000000000000, 0.000000000000000000 ) ) ;
#40077=CIRCLE ( 'NONE', #35965, 0.09999999999999982514 ) ;
#40078=AXIS2_PLACEMENT_3D ( 'NONE', #112926, #114220, #93936 ) ;
#40079=VERTEX_POINT ( 'NONE', #48040 ) ;
#40080=EDGE_CURVE ( 'NONE', #121980, #14780, #99908, .T. ) ;
#40081=DIRECTION ( 'NONE',  ( -0.000000000000000000, -1.000000000000000000, -0.000000000000000000 ) ) ;
#40082=EDGE_CURVE ( 'NONE', #127955, #69509, #35637, .T. ) ;
#40083=VERTEX_POINT ( 'NONE', #6151 ) ;
#40084=DIRECTION ( 'NONE',  ( -0.000000000000000000, -1.000000000000000000, -0.000000000000000000 ) ) ;
#40085=ORIENTED_EDGE ( 'NONE', *, *, #76416, .F. ) ;
#40086=DIRECTION ( 'NONE',  ( -0.000000000000000000, 1.000000000000000000, -0.000000000000000000 ) ) ;
#40087=ADVANCED_FACE ( 'NONE', ( #56544 ), #46098, .T. ) ;
#40088=ORIENTED_EDGE ( 'NONE', *, *, #60092, .F. ) ;
#40089=VERTEX_POINT ( 'NONE', #116115 ) ;
#40090=ADVANCED_FACE ( 'NONE', ( #40146 ), #51272, .T. ) ;
#40091=DIRECTION ( 'NONE',  ( -0.000000000000000000, -1.000000000000000000, -0.000000000000000000 ) ) ;
#40092=CARTESIAN_POINT ( 'NONE',  ( 0.7999999999999553024, 2.500000000000000000, -4.230127018922201998 ) ) ;
#40094=CARTESIAN_POINT ( 'NONE',  ( -13.54999999999998828, 2.500000000000000000, -2.511473670974875727 ) ) ;
#40096=FACE_OUTER_BOUND ( 'NONE', #12730, .T. ) ;
#40097=AXIS2_PLACEMENT_3D ( 'NONE', #111206, #121683, #60219 ) ;
#40098=DIRECTION ( 'NONE',  ( 0.000000000000000000, 0.000000000000000000, 1.000000000000000000 ) ) ;
#40099=DIRECTION ( 'NONE',  ( -4.274815082592931898E-19, -0.9999939076577903929, -0.003490651415223739937 ) ) ;
#40100=CIRCLE ( 'NONE', #69322, 0.06509327318403745899 ) ;
#40101=AXIS2_PLACEMENT_3D ( 'NONE', #115304, #6014, #25663 ) ;
#40102=FACE_OUTER_BOUND ( 'NONE', #84901, .T. ) ;
#40103=DIRECTION ( 'NONE',  ( -0.000000000000000000, 1.000000000000000000, -0.000000000000000000 ) ) ;
#40104=AXIS2_PLACEMENT_3D ( 'NONE', #69335, #41205, #100109 ) ;
#40105=ORIENTED_EDGE ( 'NONE', *, *, #82452, .T. ) ;
#40106=CIRCLE ( 'NONE', #63085, 0.06509327318403745899 ) ;
#40107=ORIENTED_EDGE ( 'NONE', *, *, #40847, .F. ) ;
#40108=EDGE_LOOP ( 'NONE', ( #21951, #31986 ) ) ;
#40109=DIRECTION ( 'NONE',  ( 0.000000000000000000, 0.000000000000000000, 1.000000000000000000 ) ) ;
#40110=CARTESIAN_POINT ( 'NONE',  ( -11.89999999999999680, 2.500000000000000000, -4.676537180435976104 ) ) ;
#40111=AXIS2_PLACEMENT_3D ( 'NONE', #19334, #68439, #69740 ) ;
#40112=DIRECTION ( 'NONE',  ( -0.000000000000000000, 1.000000000000000000, -0.000000000000000000 ) ) ;
#40113=EDGE_LOOP ( 'NONE', ( #40233, #18766, #58477, #56651 ) ) ;
#40114=FACE_BOUND ( 'NONE', #48137, .T. ) ;
#40115=ORIENTED_EDGE ( 'NONE', *, *, #104221, .F. ) ;
#40116=DIRECTION ( 'NONE',  ( 0.000000000000000000, 0.000000000000000000, -1.000000000000000000 ) ) ;
#40117=DIRECTION ( 'NONE',  ( 0.000000000000000000, 1.000000000000000000, 0.000000000000000000 ) ) ;
#40118=DIRECTION ( 'NONE',  ( -4.274815082592931898E-19, -0.9999939076577903929, -0.003490651415223739937 ) ) ;
#40119=CARTESIAN_POINT ( 'NONE',  ( 7.299999999999924327, 2.500000000000000000, 0.2464101615137735679 ) ) ;
#40120=CARTESIAN_POINT ( 'NONE',  ( 8.099999999999923261, 12.50000000000000000, 4.741630453620009789 ) ) ;
#40121=CARTESIAN_POINT ( 'NONE',  ( 6.249999999999965361, 2.500000000000000000, 2.165063509461097713 ) ) ;
#40122=DIRECTION ( 'NONE',  ( 0.000000000000000000, 1.000000000000000000, 0.000000000000000000 ) ) ;
#40123=DIRECTION ( 'NONE',  ( 0.000000000000000000, 1.000000000000000000, 0.000000000000000000 ) ) ;
#40124=DIRECTION ( 'NONE',  ( 0.000000000000000000, -0.9999939076577903929, 0.003490651415223739937 ) ) ;
#40125=ORIENTED_EDGE ( 'NONE', *, *, #49530, .T. ) ;
#40126=ORIENTED_EDGE ( 'NONE', *, *, #83385, .F. ) ;
#40127=ORIENTED_EDGE ( 'NONE', *, *, #92792, .F. ) ;
#40128=VERTEX_POINT ( 'NONE', #79437 ) ;
#40129=CARTESIAN_POINT ( 'NONE',  ( -12.49999999999995914, 2.500000000000000000, 0.1000000000000018513 ) ) ;
#40131=DIRECTION ( 'NONE',  ( -0.000000000000000000, 1.000000000000000000, -0.000000000000000000 ) ) ;
#40132=EDGE_CURVE ( 'NONE', #85147, #72947, #70249, .T. ) ;
#40133=VERTEX_POINT ( 'NONE', #60450 ) ;
#40134=ORIENTED_EDGE ( 'NONE', *, *, #51657, .F. ) ;
#40135=EDGE_LOOP ( 'NONE', ( #120855, #56282, #67009, #27980 ) ) ;
#40136=EDGE_CURVE ( 'NONE', #78385, #74255, #83187, .T. ) ;
#40137=CARTESIAN_POINT ( 'NONE',  ( -4.150000000000024336, 2.500000000000000000, 2.165063509461097713 ) ) ;
#40138=EDGE_CURVE ( 'NONE', #113689, #107267, #129264, .T. ) ;
#40139=CONICAL_SURFACE ( 'NONE', #98691, 0.1000000000000002554, 0.003490658503988666988 ) ;
#40140=AXIS2_PLACEMENT_3D ( 'NONE', #26977, #105536, #116629 ) ;
#40141=DIRECTION ( 'NONE',  ( 0.000000000000000000, 0.000000000000000000, 1.000000000000000000 ) ) ;
#40142=CARTESIAN_POINT ( 'NONE',  ( -6.900000000000015454, 12.50000000000000000, 4.611443907251934426 ) ) ;
#40143=CARTESIAN_POINT ( 'NONE',  ( 11.84999999999990727, 12.50000000000000000, -2.576566944158915184 ) ) ;
#40144=EDGE_CURVE ( 'NONE', #95427, #113919, #25056, .T. ) ;
#40145=DIRECTION ( 'NONE',  ( -0.000000000000000000, -1.000000000000000000, -0.000000000000000000 ) ) ;
#40146=FACE_OUTER_BOUND ( 'NONE', #14191, .T. ) ;
#40147=DIRECTION ( 'NONE',  ( 0.000000000000000000, 0.000000000000000000, 1.000000000000000000 ) ) ;
#40148=ORIENTED_EDGE ( 'NONE', *, *, #77901, .F. ) ;
#40149=AXIS2_PLACEMENT_3D ( 'NONE', #18798, #27984, #69178 ) ;
#40150=AXIS2_PLACEMENT_3D ( 'NONE', #31781, #80239, #122734 ) ;
#40151=DIRECTION ( 'NONE',  ( -0.000000000000000000, -1.000000000000000000, -0.000000000000000000 ) ) ;
#40153=ORIENTED_EDGE ( 'NONE', *, *, #121130, .T. ) ;
#40154=CONICAL_SURFACE ( 'NONE', #123742, 0.09999999999999999167, 0.003490658503988666988 ) ;
#40155=EDGE_CURVE ( 'NONE', #43896, #46586, #122892, .T. ) ;
#40156=ORIENTED_EDGE ( 'NONE', *, *, #73844, .T. ) ;
#40157=AXIS2_PLACEMENT_3D ( 'NONE', #3010, #23276, #63209 ) ;
#40158=EDGE_LOOP ( 'NONE', ( #36301, #118478, #43591, #114253 ) ) ;
#40159=DIRECTION ( 'NONE',  ( 0.000000000000000000, 0.000000000000000000, 1.000000000000000000 ) ) ;
#40160=EDGE_LOOP ( 'NONE', ( #81837, #92328 ) ) ;
#40161=ORIENTED_EDGE ( 'NONE', *, *, #87238, .F. ) ;
#40162=AXIS2_PLACEMENT_3D ( 'NONE', #83214, #941, #40894 ) ;
#40163=CARTESIAN_POINT ( 'NONE',  ( -11.64999999999999680, 12.50000000000000000, 2.857883832488649301 ) ) ;
#40164=AXIS2_PLACEMENT_3D ( 'NONE', #33501, #123774, #92389 ) ;
#40165=DIRECTION ( 'NONE',  ( 0.000000000000000000, 0.000000000000000000, -1.000000000000000000 ) ) ;
#40166=DIRECTION ( 'NONE',  ( 0.000000000000000000, 0.000000000000000000, -1.000000000000000000 ) ) ;
#40167=DIRECTION ( 'NONE',  ( 0.000000000000000000, 0.000000000000000000, -1.000000000000000000 ) ) ;
#40168=AXIS2_PLACEMENT_3D ( 'NONE', #30927, #117992, #78746 ) ;
#40169=AXIS2_PLACEMENT_3D ( 'NONE', #113393, #84583, #54472 ) ;
#40171=DIRECTION ( 'NONE',  ( 0.000000000000000000, 0.000000000000000000, 1.000000000000000000 ) ) ;
#40172=CIRCLE ( 'NONE', #100775, 0.06509327318403745899 ) ;
#40173=VERTEX_POINT ( 'NONE', #81370 ) ;
#40174=DIRECTION ( 'NONE',  ( 0.000000000000000000, -0.000000000000000000, 1.000000000000000000 ) ) ;
#40175=VERTEX_POINT ( 'NONE', #29676 ) ;
#40176=FACE_OUTER_BOUND ( 'NONE', #58547, .T. ) ;
#40177=VERTEX_POINT ( 'NONE', #121279 ) ;
#40179=CIRCLE ( 'NONE', #56866, 0.06509327318403745899 ) ;
#40180=CARTESIAN_POINT ( 'NONE',  ( -9.400000000000007461, 2.500000000000000000, 4.776537180435972196 ) ) ;
#40181=ORIENTED_EDGE ( 'NONE', *, *, #109575, .F. ) ;
#40183=DIRECTION ( 'NONE',  ( 0.000000000000000000, 1.000000000000000000, 0.000000000000000000 ) ) ;
#40184=ORIENTED_EDGE ( 'NONE', *, *, #120226, .F. ) ;
#40185=CARTESIAN_POINT ( 'NONE',  ( 15.59999999999988951, 12.50000000000000000, -0.3464101615137783474 ) ) ;
#40186=EDGE_LOOP ( 'NONE', ( #7634, #20086, #42176, #36277 ) ) ;
#40187=ORIENTED_EDGE ( 'NONE', *, *, #96341, .F. ) ;
#40188=PLANE ( 'NONE',  #99896 ) ;
#40189=FACE_OUTER_BOUND ( 'NONE', #96222, .T. ) ;
#40191=CARTESIAN_POINT ( 'NONE',  ( -10.40000000000000213, 12.50000000000000000, 4.330127018922196314 ) ) ;
#40192=CARTESIAN_POINT ( 'NONE',  ( -1.650000000000035660, 2.500000000000000000, 7.188010851410848723 ) ) ;
#40193=EDGE_CURVE ( 'NONE', #125178, #75848, #41433, .T. ) ;
#40194=ORIENTED_EDGE ( 'NONE', *, *, #68310, .T. ) ;
#40195=CARTESIAN_POINT ( 'NONE',  ( 12.89999999999989910, 2.500000000000000000, 0.7928203230275495672 ) ) ;
#40196=AXIS2_PLACEMENT_3D ( 'NONE', #54714, #92065, #63259 ) ;
#40197=AXIS2_PLACEMENT_3D ( 'NONE', #109996, #109343, #110632 ) ;
#40199=ORIENTED_EDGE ( 'NONE', *, *, #45858, .T. ) ;
#40200=FACE_OUTER_BOUND ( 'NONE', #104715, .T. ) ;
#40201=CARTESIAN_POINT ( 'NONE',  ( -8.150000000000009237, 2.500000000000000000, 6.841600689897072485 ) ) ;
#40202=AXIS2_PLACEMENT_3D ( 'NONE', #122460, #114544, #51779 ) ;
#40203=AXIS2_PLACEMENT_3D ( 'NONE', #117220, #23891, #27558 ) ;
#40204=AXIS2_PLACEMENT_3D ( 'NONE', #95187, #45453, #55266 ) ;
#40205=CIRCLE ( 'NONE', #56896, 0.1000000000000002554 ) ;
#40207=CARTESIAN_POINT ( 'NONE',  ( -14.79999999999998295, 12.50000000000000000, -0.3464101615137760715 ) ) ;
#40208=LINE ( 'NONE', #58564, #96630 ) ;
#40209=FACE_OUTER_BOUND ( 'NONE', #106913, .T. ) ;
#40210=LINE ( 'NONE', #87988, #97701 ) ;
#40211=VERTEX_POINT ( 'NONE', #8718 ) ;
#40212=VECTOR ( 'NONE', #100686, 1000.000000000000000 ) ;
#40213=CARTESIAN_POINT ( 'NONE',  ( -11.24999999999999822, 2.500000000000000000, 5.902370205355745192 ) ) ;
#40214=DIRECTION ( 'NONE',  ( 0.000000000000000000, 0.000000000000000000, -1.000000000000000000 ) ) ;
#40216=ORIENTED_EDGE ( 'NONE', *, *, #5794, .F. ) ;
#40217=DIRECTION ( 'NONE',  ( 0.000000000000000000, 0.000000000000000000, 1.000000000000000000 ) ) ;
#40218=ORIENTED_EDGE ( 'NONE', *, *, #99982, .F. ) ;
#40219=ORIENTED_EDGE ( 'NONE', *, *, #26190, .F. ) ;
#40220=CARTESIAN_POINT ( 'NONE',  ( 8.949999999999921130, 2.500000000000000000, 1.918653347947321564 ) ) ;
#40221=ORIENTED_EDGE ( 'NONE', *, *, #25814, .F. ) ;
#40222=DIRECTION ( 'NONE',  ( 0.000000000000000000, 0.000000000000000000, -1.000000000000000000 ) ) ;
#40223=CARTESIAN_POINT ( 'NONE',  ( 4.599999999999937472, 2.500000000000000000, 0.7928203230275495672 ) ) ;
#40224=CIRCLE ( 'NONE', #105046, 0.06509327318403745899 ) ;
#40225=VERTEX_POINT ( 'NONE', #80721 ) ;
#40226=EDGE_CURVE ( 'NONE', #20798, #42905, #1493, .T. ) ;
#40227=DIRECTION ( 'NONE',  ( 0.000000000000000000, -0.000000000000000000, 1.000000000000000000 ) ) ;
#40228=CARTESIAN_POINT ( 'NONE',  ( -9.350000000000006750, 2.500000000000000000, 1.918653347947321564 ) ) ;
#40229=DIRECTION ( 'NONE',  ( -0.000000000000000000, -1.000000000000000000, -0.000000000000000000 ) ) ;
#40230=ADVANCED_FACE ( 'NONE', ( #128551 ), #71523, .T. ) ;
#40231=AXIS2_PLACEMENT_3D ( 'NONE', #110255, #123141, #83221 ) ;
#40232=EDGE_CURVE ( 'NONE', #21808, #115792, #104104, .T. ) ;
#40233=ORIENTED_EDGE ( 'NONE', *, *, #48962, .F. ) ;
#40235=ORIENTED_EDGE ( 'NONE', *, *, #57877, .F. ) ;
#40236=ORIENTED_EDGE ( 'NONE', *, *, #34029, .T. ) ;
#40237=DIRECTION ( 'NONE',  ( 0.000000000000000000, 0.000000000000000000, 1.000000000000000000 ) ) ;
#40239=EDGE_CURVE ( 'NONE', #19953, #40728, #108863, .T. ) ;
#40240=EDGE_CURVE ( 'NONE', #128103, #79041, #119336, .T. ) ;
#40241=FACE_OUTER_BOUND ( 'NONE', #86462, .T. ) ;
#40243=FACE_BOUND ( 'NONE', #46332, .T. ) ;
#40244=ORIENTED_EDGE ( 'NONE', *, *, #98125, .T. ) ;
#40245=ADVANCED_FACE ( 'NONE', ( #39526 ), #109531, .T. ) ;
#40246=EDGE_CURVE ( 'NONE', #23183, #6037, #33557, .T. ) ;
#40247=CARTESIAN_POINT ( 'NONE',  ( 5.599999999999934808, 12.50000000000000000, -4.676537180435978769 ) ) ;
#40248=DIRECTION ( 'NONE',  ( 0.000000000000000000, 1.000000000000000000, 0.000000000000000000 ) ) ;
#40249=VECTOR ( 'NONE', #92888, 1000.000000000000000 ) ;
#40250=EDGE_LOOP ( 'NONE', ( #2402, #49653, #89383, #78339 ) ) ;
#40251=CONICAL_SURFACE ( 'NONE', #115524, 0.1000000000000002554, 0.003490658503988666988 ) ;
#40253=CARTESIAN_POINT ( 'NONE',  ( 13.54999999999989768, 12.50000000000000000, -2.511473670974877948 ) ) ;
#40254=CONICAL_SURFACE ( 'NONE', #71637, 0.1000000000000002554, 0.003490658503988666988 ) ;
#40255=AXIS2_PLACEMENT_3D ( 'NONE', #11814, #59668, #71366 ) ;
#40257=LINE ( 'NONE', #108961, #79980 ) ;
#40258=CARTESIAN_POINT ( 'NONE',  ( 9.799999999999915445, 12.50000000000000000, 4.048810130592458201 ) ) ;
#40259=CARTESIAN_POINT ( 'NONE',  ( 10.64999999999991331, 2.500000000000000000, 6.741600689897071952 ) ) ;
#40260=ADVANCED_FACE ( 'NONE', ( #52538 ), #14200, .T. ) ;
#40261=CARTESIAN_POINT ( 'NONE',  ( -13.09999999999999076, 2.500000000000000000, 4.576537180435972019 ) ) ;
#40262=CONICAL_SURFACE ( 'NONE', #77889, 0.09999999999999982514, 0.003490658503988666988 ) ;
#40263=DIRECTION ( 'NONE',  ( 0.000000000000000000, 1.000000000000000000, 0.000000000000000000 ) ) ;
#40264=VERTEX_POINT ( 'NONE', #34851 ) ;
#40265=AXIS2_PLACEMENT_3D ( 'NONE', #3875, #34658, #24170 ) ;
#40266=VERTEX_POINT ( 'NONE', #114039 ) ;
#40267=ORIENTED_EDGE ( 'NONE', *, *, #46600, .F. ) ;
#40268=EDGE_LOOP ( 'NONE', ( #19776, #91056, #84646, #108472 ) ) ;
#40269=CARTESIAN_POINT ( 'NONE',  ( 6.649999999999928413, 2.500000000000000000, 2.757883832488649656 ) ) ;
#40270=CARTESIAN_POINT ( 'NONE',  ( 8.749999999999953815, 2.500000000000000000, 6.495190528383297135 ) ) ;
#40271=EDGE_LOOP ( 'NONE', ( #42473, #50890, #104009, #36338 ) ) ;
#40272=FACE_BOUND ( 'NONE', #106643, .T. ) ;
#40273=DIRECTION ( 'NONE',  ( 0.000000000000000000, -0.9999939076577903929, 0.003490651415223739937 ) ) ;
#40274=DIRECTION ( 'NONE',  ( 0.000000000000000000, 0.000000000000000000, -1.000000000000000000 ) ) ;
#40275=CARTESIAN_POINT ( 'NONE',  ( -1.050000000000038236, 12.50000000000000000, -6.148780366869526226 ) ) ;
#40276=CARTESIAN_POINT ( 'NONE',  ( 11.04999999999990834, 12.50000000000000000, -6.841600689897077814 ) ) ;
#40277=CARTESIAN_POINT ( 'NONE',  ( -8.550000000000011369, 12.50000000000000000, 1.818653347947321475 ) ) ;
#40278=DIRECTION ( 'NONE',  ( 0.000000000000000000, 0.000000000000000000, 1.000000000000000000 ) ) ;
#40279=AXIS2_PLACEMENT_3D ( 'NONE', #64323, #44046, #123875 ) ;
#40280=CARTESIAN_POINT ( 'NONE',  ( 3.749999999999975131, 2.500000000000000000, 6.495190528383297135 ) ) ;
#40281=ORIENTED_EDGE ( 'NONE', *, *, #19491, .F. ) ;
#40282=ORIENTED_EDGE ( 'NONE', *, *, #102585, .F. ) ;
#40283=ORIENTED_EDGE ( 'NONE', *, *, #71727, .T. ) ;
#40284=EDGE_LOOP ( 'NONE', ( #61722, #201, #51639, #127305 ) ) ;
#40285=ORIENTED_EDGE ( 'NONE', *, *, #60858, .T. ) ;
#40286=CONICAL_SURFACE ( 'NONE', #88276, 0.1000000000000002554, 0.003490658503988666988 ) ;
#40288=AXIS2_PLACEMENT_3D ( 'NONE', #31443, #92942, #54291 ) ;
#40289=AXIS2_PLACEMENT_3D ( 'NONE', #46433, #90057, #66076 ) ;
#40290=EDGE_CURVE ( 'NONE', #40089, #2945, #53197, .T. ) ;
#40291=CARTESIAN_POINT ( 'NONE',  ( -5.650000000000019895, 2.500000000000000000, 6.941600689897073018 ) ) ;
#40292=CARTESIAN_POINT ( 'NONE',  ( -5.850000000000018296, 12.50000000000000000, 7.122917578226811486 ) ) ;
#40293=EDGE_CURVE ( 'NONE', #102428, #45275, #5878, .T. ) ;
#40294=VERTEX_POINT ( 'NONE', #2789 ) ;
#40295=DIRECTION ( 'NONE',  ( 0.000000000000000000, 1.000000000000000000, 0.000000000000000000 ) ) ;
#40296=ADVANCED_FACE ( 'NONE', ( #62372 ), #95782, .T. ) ;
#40297=AXIS2_PLACEMENT_3D ( 'NONE', #73838, #83666, #71251 ) ;
#40298=ADVANCED_FACE ( 'NONE', ( #81989 ), #94382, .T. ) ;
#40299=AXIS2_PLACEMENT_3D ( 'NONE', #14723, #54652, #85419 ) ;
#40300=CARTESIAN_POINT ( 'NONE',  ( 1.849999999999950129, 2.500000000000000000, -6.841600689897078702 ) ) ;
#40302=DIRECTION ( 'NONE',  ( 0.000000000000000000, 0.000000000000000000, -1.000000000000000000 ) ) ;
#40303=CARTESIAN_POINT ( 'NONE',  ( -15.19999999999998153, 2.500000000000000000, -0.3464101615137759604 ) ) ;
#40304=CIRCLE ( 'NONE', #109228, 0.06509327318403741736 ) ;
#40305=CIRCLE ( 'NONE', #29833, 0.06509327318403745899 ) ;
#40306=EDGE_CURVE ( 'NONE', #85331, #79392, #43476, .T. ) ;
#40307=ORIENTED_EDGE ( 'NONE', *, *, #50024, .F. ) ;
#40308=DIRECTION ( 'NONE',  ( -0.000000000000000000, -1.000000000000000000, -0.000000000000000000 ) ) ;
#40309=AXIS2_PLACEMENT_3D ( 'NONE', #101839, #122769, #71736 ) ;
#40310=ADVANCED_FACE ( 'NONE', ( #32282 ), #127102, .T. ) ;
#40312=ORIENTED_EDGE ( 'NONE', *, *, #22047, .T. ) ;
#40313=EDGE_CURVE ( 'NONE', #98576, #91821, #93119, .T. ) ;
#40314=EDGE_LOOP ( 'NONE', ( #163, #72333, #15045, #21408 ) ) ;
#40315=FACE_OUTER_BOUND ( 'NONE', #75588, .T. ) ;
#40316=DIRECTION ( 'NONE',  ( 0.000000000000000000, -0.9999939076577903929, 0.003490651415223739937 ) ) ;
#40317=DIRECTION ( 'NONE',  ( -0.000000000000000000, -1.000000000000000000, -0.000000000000000000 ) ) ;
#40318=ORIENTED_EDGE ( 'NONE', *, *, #40313, .T. ) ;
#40319=EDGE_CURVE ( 'NONE', #60096, #37015, #91819, .T. ) ;
#40320=VERTEX_POINT ( 'NONE', #23731 ) ;
#40321=CONICAL_SURFACE ( 'NONE', #102988, 0.1000000000000000472, 0.003490658503988666988 ) ;
#40322=DIRECTION ( 'NONE',  ( 0.000000000000000000, 0.000000000000000000, 1.000000000000000000 ) ) ;
#40323=DIRECTION ( 'NONE',  ( 0.000000000000000000, 0.000000000000000000, 1.000000000000000000 ) ) ;
#40324=FACE_OUTER_BOUND ( 'NONE', #127264, .T. ) ;
#40325=FACE_OUTER_BOUND ( 'NONE', #59859, .T. ) ;
#40326=ORIENTED_EDGE ( 'NONE', *, *, #117363, .F. ) ;
#40327=DIRECTION ( 'NONE',  ( 0.000000000000000000, 1.000000000000000000, 0.000000000000000000 ) ) ;
#40328=AXIS2_PLACEMENT_3D ( 'NONE', #36836, #46645, #99464 ) ;
#40329=ORIENTED_EDGE ( 'NONE', *, *, #84151, .F. ) ;
#40330=PLANE ( 'NONE',  #116759 ) ;
#40331=AXIS2_PLACEMENT_3D ( 'NONE', #76311, #126702, #37033 ) ;
#40332=CONICAL_SURFACE ( 'NONE', #115508, 0.09999999999999999167, 0.003490658503988666988 ) ;
#40334=DIRECTION ( 'NONE',  ( -0.000000000000000000, 1.000000000000000000, -0.000000000000000000 ) ) ;
#40335=DIRECTION ( 'NONE',  ( 0.000000000000000000, 1.000000000000000000, 0.000000000000000000 ) ) ;
#40336=FACE_OUTER_BOUND ( 'NONE', #122515, .T. ) ;
#40337=EDGE_CURVE ( 'NONE', #67756, #95287, #64715, .T. ) ;
#40338=DIRECTION ( 'NONE',  ( 0.000000000000000000, 1.000000000000000000, 0.000000000000000000 ) ) ;
#40339=AXIS2_PLACEMENT_3D ( 'NONE', #87710, #96238, #26870 ) ;
#40342=AXIS2_PLACEMENT_3D ( 'NONE', #56369, #17056, #126410 ) ;
#40343=CARTESIAN_POINT ( 'NONE',  ( 7.899999999999924860, 2.500000000000000000, 4.230127018922196669 ) ) ;
#40344=AXIS2_PLACEMENT_3D ( 'NONE', #17808, #97667, #77388 ) ;
#40345=CARTESIAN_POINT ( 'NONE',  ( 17.50000000000000000, -2.500000000000000000, 4.000000000000001776 ) ) ;
#40346=ORIENTED_EDGE ( 'NONE', *, *, #18456, .T. ) ;
#40347=ORIENTED_EDGE ( 'NONE', *, *, #32351, .T. ) ;
#40348=ORIENTED_EDGE ( 'NONE', *, *, #111197, .F. ) ;
#40349=CARTESIAN_POINT ( 'NONE',  ( -5.850000000000019185, 12.50000000000000000, 2.165063509461097713 ) ) ;
#40350=DIRECTION ( 'NONE',  ( 0.000000000000000000, 0.000000000000000000, 1.000000000000000000 ) ) ;
#40351=LINE ( 'NONE', #39723, #21907 ) ;
#40353=CIRCLE ( 'NONE', #73773, 0.06509327318403745899 ) ;
#40354=DIRECTION ( 'NONE',  ( 0.000000000000000000, 1.000000000000000000, 0.000000000000000000 ) ) ;
#40355=LINE ( 'NONE', #1689, #571 ) ;
#40356=CIRCLE ( 'NONE', #96466, 0.06509327318403745899 ) ;
#40357=CARTESIAN_POINT ( 'NONE',  ( -1.850000000000033840, 12.50000000000000000, 2.576566944158910744 ) ) ;
#40358=EDGE_CURVE ( 'NONE', #88083, #20150, #85648, .T. ) ;
#40359=CONICAL_SURFACE ( 'NONE', #52863, 0.1000000000000000056, 0.003490658503988666988 ) ;
#40360=CARTESIAN_POINT ( 'NONE',  ( -11.84999999999999609, 2.500000000000000000, 6.841600689897072485 ) ) ;
#40361=VECTOR ( 'NONE', #48369, 1000.000000000000000 ) ;
#40362=CIRCLE ( 'NONE', #44449, 0.1000000000000002554 ) ;
#40363=DIRECTION ( 'NONE',  ( 0.000000000000000000, 1.000000000000000000, 0.000000000000000000 ) ) ;
#40364=VECTOR ( 'NONE', #56653, 1000.000000000000000 ) ;
#40365=ORIENTED_EDGE ( 'NONE', *, *, #98264, .T. ) ;
#40366=FACE_OUTER_BOUND ( 'NONE', #68629, .T. ) ;
#40367=EDGE_CURVE ( 'NONE', #103425, #21203, #127514, .T. ) ;
#40368=CARTESIAN_POINT ( 'NONE',  ( 9.349999999999919709, 12.50000000000000000, 2.511473670974873507 ) ) ;
#40369=FACE_OUTER_BOUND ( 'NONE', #17785, .T. ) ;
#40370=CARTESIAN_POINT ( 'NONE',  ( -2.900000000000029665, 2.500000000000000000, 3.637306695894644726 ) ) ;
#40371=CARTESIAN_POINT ( 'NONE',  ( -1.650000000000035660, 12.50000000000000000, 7.253104124594885960 ) ) ;
#40372=VERTEX_POINT ( 'NONE', #104210 ) ;
#40373=CARTESIAN_POINT ( 'NONE',  ( -7.700000000000014388, 12.50000000000000000, -0.4115034346978156399 ) ) ;
#40374=FACE_OUTER_BOUND ( 'NONE', #104155, .T. ) ;
#40375=DIRECTION ( 'NONE',  ( -4.274815082592931898E-19, -0.9999939076577903929, -0.003490651415223739937 ) ) ;
#40376=ORIENTED_EDGE ( 'NONE', *, *, #78366, .T. ) ;
#40377=CIRCLE ( 'NONE', #113517, 0.1000000000000000472 ) ;
#40378=AXIS2_PLACEMENT_3D ( 'NONE', #120371, #81715, #121640 ) ;
#40379=VERTEX_POINT ( 'NONE', #84574 ) ;
#40380=LINE ( 'NONE', #60028, #111616 ) ;
#40381=CIRCLE ( 'NONE', #88677, 0.1000000000000002554 ) ;
#40382=EDGE_LOOP ( 'NONE', ( #38615, #84162 ) ) ;
#40383=AXIS2_PLACEMENT_3D ( 'NONE', #109969, #20291, #100151 ) ;
#40384=ORIENTED_EDGE ( 'NONE', *, *, #8458, .T. ) ;
#40385=CARTESIAN_POINT ( 'NONE',  ( 6.449999999999933564, 12.50000000000000000, -6.906693963081115939 ) ) ;
#40386=AXIS2_PLACEMENT_3D ( 'NONE', #77780, #18869, #118361 ) ;
#40387=AXIS2_PLACEMENT_3D ( 'NONE', #57237, #48722, #29711 ) ;
#40388=CARTESIAN_POINT ( 'NONE',  ( 19.08853762629022199, 0.5565172524007554467, -4.470057054643568506 ) ) ;
#40389=DIRECTION ( 'NONE',  ( -0.000000000000000000, -1.000000000000000000, -0.000000000000000000 ) ) ;
#40391=AXIS2_PLACEMENT_3D ( 'NONE', #120533, #53082, #1390 ) ;
#40392=EDGE_LOOP ( 'NONE', ( #36859, #94790 ) ) ;
#40393=AXIS2_PLACEMENT_3D ( 'NONE', #99285, #89455, #107808 ) ;
#40394=CIRCLE ( 'NONE', #65500, 0.1000000000000002554 ) ;
#40395=EDGE_CURVE ( 'NONE', #110679, #109560, #54463, .T. ) ;
#40396=DIRECTION ( 'NONE',  ( -0.000000000000000000, 1.000000000000000000, -0.000000000000000000 ) ) ;
#40397=AXIS2_PLACEMENT_3D ( 'NONE', #44314, #15490, #86153 ) ;
#40398=EDGE_LOOP ( 'NONE', ( #69341, #59129, #106683, #67230 ) ) ;
#40399=PLANE ( 'NONE',  #95670 ) ;
#40400=CIRCLE ( 'NONE', #71781, 0.06509327318403745899 ) ;
#40401=CARTESIAN_POINT ( 'NONE',  ( -12.09999999999999609, 2.500000000000000000, 0.6928203230275535862 ) ) ;
#40402=CARTESIAN_POINT ( 'NONE',  ( 7.049999999999928768, 2.500000000000000000, -2.065063509461102065 ) ) ;
#40403=EDGE_CURVE ( 'NONE', #127796, #91980, #124512, .T. ) ;
#40404=ORIENTED_EDGE ( 'NONE', *, *, #48811, .T. ) ;
#40405=ORIENTED_EDGE ( 'NONE', *, *, #42404, .T. ) ;
#40406=ORIENTED_EDGE ( 'NONE', *, *, #124911, .T. ) ;
#40408=ORIENTED_EDGE ( 'NONE', *, *, #128325, .F. ) ;
#40410=CARTESIAN_POINT ( 'NONE',  ( 16.56576425165006583, 2.500000000000000000, 6.084390597445811899 ) ) ;
#40411=EDGE_CURVE ( 'NONE', #123530, #32792, #52205, .T. ) ;
#40412=EDGE_CURVE ( 'NONE', #95641, #31177, #106147, .T. ) ;
#40413=LINE ( 'NONE', #128802, #60817 ) ;
#40414=EDGE_CURVE ( 'NONE', #13317, #3943, #68921, .T. ) ;
#40415=FACE_BOUND ( 'NONE', #20335, .T. ) ;
#40416=EDGE_CURVE ( 'NONE', #13662, #7603, #96311, .T. ) ;
#40417=CARTESIAN_POINT ( 'NONE',  ( -3.550000000000027356, 2.500000000000000000, -2.511473670974877948 ) ) ;
#40418=CARTESIAN_POINT ( 'NONE',  ( 8.949999999999917577, 2.500000000000000000, 6.148780366869520009 ) ) ;
#40419=DIRECTION ( 'NONE',  ( -0.000000000000000000, 1.000000000000000000, -0.000000000000000000 ) ) ;
#40420=CARTESIAN_POINT ( 'NONE',  ( -10.84999999999999964, 2.500000000000000000, 7.288010851410849256 ) ) ;
#40421=AXIS2_PLACEMENT_3D ( 'NONE', #58432, #9960, #40070 ) ;
#40422=DIRECTION ( 'NONE',  ( 0.000000000000000000, 0.000000000000000000, -1.000000000000000000 ) ) ;
#40423=DIRECTION ( 'NONE',  ( -0.000000000000000000, -1.000000000000000000, -0.000000000000000000 ) ) ;
#40424=EDGE_CURVE ( 'NONE', #3575, #12586, #12485, .T. ) ;
#40425=LINE ( 'NONE', #118316, #61729 ) ;
#40426=CONICAL_SURFACE ( 'NONE', #113566, 0.09999999999999982514, 0.003490658503988666988 ) ;
#40427=AXIS2_PLACEMENT_3D ( 'NONE', #26418, #66323, #4814 ) ;
#40428=ADVANCED_FACE ( 'NONE', ( #125761 ), #110773, .T. ) ;
#40429=CIRCLE ( 'NONE', #98989, 0.06509327318403745899 ) ;
#40430=EDGE_CURVE ( 'NONE', #27399, #66014, #54345, .T. ) ;
#40431=FACE_OUTER_BOUND ( 'NONE', #113421, .T. ) ;
#40432=ORIENTED_EDGE ( 'NONE', *, *, #95730, .F. ) ;
#40433=ORIENTED_EDGE ( 'NONE', *, *, #77516, .T. ) ;
#40434=EDGE_LOOP ( 'NONE', ( #92150, #110221, #27652, #34043 ) ) ;
#40435=EDGE_LOOP ( 'NONE', ( #104110, #62196 ) ) ;
#40436=DIRECTION ( 'NONE',  ( -0.000000000000000000, 1.000000000000000000, -0.000000000000000000 ) ) ;
#40437=CARTESIAN_POINT ( 'NONE',  ( 9.349999999999916156, 12.50000000000000000, 6.083687093685482772 ) ) ;
#40438=FACE_BOUND ( 'NONE', #27448, .T. ) ;
#40439=AXIS2_PLACEMENT_3D ( 'NONE', #3221, #52312, #21564 ) ;
#40440=CIRCLE ( 'NONE', #59219, 0.1000000000000000472 ) ;
#40441=DIRECTION ( 'NONE',  ( 0.000000000000000000, 0.000000000000000000, 1.000000000000000000 ) ) ;
#40442=CONICAL_SURFACE ( 'NONE', #113585, 0.1000000000000002554, 0.003490658503988666988 ) ;
#40443=VERTEX_POINT ( 'NONE', #95691 ) ;
#40444=CARTESIAN_POINT ( 'NONE',  ( 11.89999999999990798, 2.500000000000000000, -4.676537180435977881 ) ) ;
#40445=DIRECTION ( 'NONE',  ( 0.000000000000000000, 0.000000000000000000, -1.000000000000000000 ) ) ;
#40446=DIRECTION ( 'NONE',  ( -0.000000000000000000, 1.000000000000000000, -0.000000000000000000 ) ) ;
#40447=DIRECTION ( 'NONE',  ( 0.000000000000000000, 1.000000000000000000, 0.000000000000000000 ) ) ;
#40448=ORIENTED_EDGE ( 'NONE', *, *, #53814, .F. ) ;
#40449=DIRECTION ( 'NONE',  ( 0.000000000000000000, 0.000000000000000000, 1.000000000000000000 ) ) ;
#40450=AXIS2_PLACEMENT_3D ( 'NONE', #32375, #43465, #72279 ) ;
#40451=AXIS2_PLACEMENT_3D ( 'NONE', #55937, #105028, #114847 ) ;
#40452=AXIS2_PLACEMENT_3D ( 'NONE', #19517, #59482, #129510 ) ;
#40453=VERTEX_POINT ( 'NONE', #57030 ) ;
#40454=VERTEX_POINT ( 'NONE', #117225 ) ;
#40455=DIRECTION ( 'NONE',  ( 0.000000000000000000, 0.000000000000000000, 1.000000000000000000 ) ) ;
#40456=DIRECTION ( 'NONE',  ( 0.000000000000000000, 0.000000000000000000, -1.000000000000000000 ) ) ;
#40457=VECTOR ( 'NONE', #90647, 1000.000000000000000 ) ;
#40458=ORIENTED_EDGE ( 'NONE', *, *, #89171, .F. ) ;
#40459=DIRECTION ( 'NONE',  ( 0.000000000000000000, 0.000000000000000000, -1.000000000000000000 ) ) ;
#40460=DIRECTION ( 'NONE',  ( 0.000000000000000000, 0.000000000000000000, 1.000000000000000000 ) ) ;
#40461=PLANE ( 'NONE',  #72440 ) ;
#40462=VERTEX_POINT ( 'NONE', #36124 ) ;
#40463=DIRECTION ( 'NONE',  ( 0.000000000000000000, 1.000000000000000000, 0.000000000000000000 ) ) ;
#40464=EDGE_CURVE ( 'NONE', #7910, #8844, #66854, .T. ) ;
#40465=VERTEX_POINT ( 'NONE', #15819 ) ;
#40466=CARTESIAN_POINT ( 'NONE',  ( -7.900000000000014566, 12.50000000000000000, -5.022947341949754119 ) ) ;
#40467=EDGE_CURVE ( 'NONE', #125626, #7881, #127088, .T. ) ;
#40468=EDGE_LOOP ( 'NONE', ( #27635, #113269 ) ) ;
#40469=DIRECTION ( 'NONE',  ( -0.000000000000000000, 1.000000000000000000, -0.000000000000000000 ) ) ;
#40470=EDGE_CURVE ( 'NONE', #70629, #96127, #100328, .T. ) ;
#40471=ORIENTED_EDGE ( 'NONE', *, *, #114967, .F. ) ;
#40472=CARTESIAN_POINT ( 'NONE',  ( -11.64999999999999680, 2.500000000000000000, -7.188010851410850499 ) ) ;
#40473=DIRECTION ( 'NONE',  ( 0.000000000000000000, -0.000000000000000000, 1.000000000000000000 ) ) ;
#40474=AXIS2_PLACEMENT_3D ( 'NONE', #103423, #34035, #32773 ) ;
#40475=DIRECTION ( 'NONE',  ( 0.000000000000000000, 0.000000000000000000, 1.000000000000000000 ) ) ;
#40476=CONICAL_SURFACE ( 'NONE', #94733, 0.1000000000000002554, 0.003490658503988666988 ) ;
#40477=DIRECTION ( 'NONE',  ( 0.000000000000000000, 0.000000000000000000, 1.000000000000000000 ) ) ;
#40478=CARTESIAN_POINT ( 'NONE',  ( 12.69999999999990337, 12.50000000000000000, -4.676537180435978769 ) ) ;
#40479=ORIENTED_EDGE ( 'NONE', *, *, #98224, .F. ) ;
#40480=ADVANCED_FACE ( 'NONE', ( #96963 ), #56396, .T. ) ;
#40481=EDGE_LOOP ( 'NONE', ( #86819, #684, #94763, #28276 ) ) ;
#40482=ORIENTED_EDGE ( 'NONE', *, *, #99721, .T. ) ;
#40483=CARTESIAN_POINT ( 'NONE',  ( -9.400000000000007461, 12.50000000000000000, -0.4115034346978157509 ) ) ;
#40484=CIRCLE ( 'NONE', #17356, 0.06509327318403745899 ) ;
#40485=AXIS2_PLACEMENT_3D ( 'NONE', #19055, #59008, #21006 ) ;
#40486=CARTESIAN_POINT ( 'NONE',  ( -5.450000000000023270, 2.500000000000000000, -6.595190528383302109 ) ) ;
#40487=AXIS2_PLACEMENT_3D ( 'NONE', #113707, #103244, #1169 ) ;
#40488=AXIS2_PLACEMENT_3D ( 'NONE', #112145, #90559, #22496 ) ;
#40489=DIRECTION ( 'NONE',  ( 0.000000000000000000, 0.000000000000000000, 1.000000000000000000 ) ) ;
#40490=VERTEX_POINT ( 'NONE', #5357 ) ;
#40491=VERTEX_POINT ( 'NONE', #26309 ) ;
#40492=ORIENTED_EDGE ( 'NONE', *, *, #64285, .T. ) ;
#40493=FACE_OUTER_BOUND ( 'NONE', #55456, .T. ) ;
#40494=VERTEX_POINT ( 'NONE', #67480 ) ;
#40495=DIRECTION ( 'NONE',  ( 0.000000000000000000, 0.000000000000000000, -1.000000000000000000 ) ) ;
#40496=CIRCLE ( 'NONE', #96893, 0.06509327318403745899 ) ;
#40497=CIRCLE ( 'NONE', #65499, 0.06509327318403745899 ) ;
#40498=AXIS2_PLACEMENT_3D ( 'NONE', #27050, #54554, #116065 ) ;
#40500=FACE_OUTER_BOUND ( 'NONE', #38226, .T. ) ;
#40501=CARTESIAN_POINT ( 'NONE',  ( -6.900000000000019007, 2.500000000000000000, -3.883716857408426648 ) ) ;
#40502=DIRECTION ( 'NONE',  ( 0.000000000000000000, 0.000000000000000000, 1.000000000000000000 ) ) ;
#40504=CARTESIAN_POINT ( 'NONE',  ( 12.09999999999990550, 2.500000000000000000, -5.022947341949754119 ) ) ;
#40505=ADVANCED_FACE ( 'NONE', ( #66210 ), #17751, .T. ) ;
#40506=LINE ( 'NONE', #70584, #8095 ) ;
#40507=VERTEX_POINT ( 'NONE', #127714 ) ;
#40508=ORIENTED_EDGE ( 'NONE', *, *, #72059, .F. ) ;
#40509=LINE ( 'NONE', #88267, #34074 ) ;
#40510=CARTESIAN_POINT ( 'NONE',  ( 7.949999999999925571, 12.50000000000000000, 2.165063509461097713 ) ) ;
#40511=ORIENTED_EDGE ( 'NONE', *, *, #55927, .F. ) ;
#40512=EDGE_LOOP ( 'NONE', ( #30148, #67151 ) ) ;
#40514=DIRECTION ( 'NONE',  ( 0.000000000000000000, 0.000000000000000000, 1.000000000000000000 ) ) ;
#40515=CARTESIAN_POINT ( 'NONE',  ( 21.23528140090950700, 2.699413673072311948, 2.293764360948889802 ) ) ;
#40516=CIRCLE ( 'NONE', #768, 0.06509327318403745899 ) ;
#40517=CARTESIAN_POINT ( 'NONE',  ( -4.350000000000023626, 12.50000000000000000, -2.576566944158915184 ) ) ;
#40518=CARTESIAN_POINT ( 'NONE',  ( -8.750000000000012434, 12.50000000000000000, -5.802370205355744659 ) ) ;
#40519=EDGE_CURVE ( 'NONE', #66127, #107210, #77969, .T. ) ;
#40520=CARTESIAN_POINT ( 'NONE',  ( 10.84999999999990905, 2.500000000000000000, -6.495190528383302464 ) ) ;
#40521=DIRECTION ( 'NONE',  ( -0.000000000000000000, -1.000000000000000000, -0.000000000000000000 ) ) ;
#40522=AXIS2_PLACEMENT_3D ( 'NONE', #4281, #93985, #125378 ) ;
#40523=FACE_OUTER_BOUND ( 'NONE', #49829, .T. ) ;
#40524=VECTOR ( 'NONE', #122524, 1000.000000000000000 ) ;
#40525=ORIENTED_EDGE ( 'NONE', *, *, #121529, .F. ) ;
#40526=CONICAL_SURFACE ( 'NONE', #48832, 0.09999999999999982514, 0.003490658503988666988 ) ;
#40527=ORIENTED_EDGE ( 'NONE', *, *, #12243, .T. ) ;
#40528=VERTEX_POINT ( 'NONE', #15158 ) ;
#40529=EDGE_LOOP ( 'NONE', ( #58012, #96314 ) ) ;
#40531=ORIENTED_EDGE ( 'NONE', *, *, #43252, .F. ) ;
#40532=AXIS2_PLACEMENT_3D ( 'NONE', #111720, #82916, #42343 ) ;
#40533=DIRECTION ( 'NONE',  ( 0.000000000000000000, 1.000000000000000000, 0.000000000000000000 ) ) ;
#40534=CARTESIAN_POINT ( 'NONE',  ( -2.900000000000030109, 2.500000000000000000, 0.5928203230275495006 ) ) ;
#40535=AXIS2_PLACEMENT_3D ( 'NONE', #38886, #96460, #46097 ) ;
#40536=ORIENTED_EDGE ( 'NONE', *, *, #75814, .F. ) ;
#40537=DIRECTION ( 'NONE',  ( -0.000000000000000000, 1.000000000000000000, -0.000000000000000000 ) ) ;
#40538=AXIS2_PLACEMENT_3D ( 'NONE', #85438, #54669, #84793 ) ;
#40539=DIRECTION ( 'NONE',  ( 0.000000000000000000, 0.000000000000000000, 1.000000000000000000 ) ) ;
#40540=DIRECTION ( 'NONE',  ( 0.000000000000000000, 0.000000000000000000, 1.000000000000000000 ) ) ;
#40542=VERTEX_POINT ( 'NONE', #35485 ) ;
#40543=ADVANCED_FACE ( 'NONE', ( #75382 ), #48011, .T. ) ;
#40544=CARTESIAN_POINT ( 'NONE',  ( 5.849999999999933920, 12.50000000000000000, -2.165063509461101710 ) ) ;
#40545=CONICAL_SURFACE ( 'NONE', #4993, 0.09999999999999982514, 0.003490658503988666988 ) ;
#40546=DIRECTION ( 'NONE',  ( 0.000000000000000000, -0.000000000000000000, 1.000000000000000000 ) ) ;
#40547=ORIENTED_EDGE ( 'NONE', *, *, #30336, .F. ) ;
#40548=VECTOR ( 'NONE', #20430, 1000.000000000000000 ) ;
#40549=CONICAL_SURFACE ( 'NONE', #9129, 0.09999999999999999167, 0.003490658503988666988 ) ;
#40550=CONICAL_SURFACE ( 'NONE', #111533, 0.1000000000000002554, 0.003490658503988666988 ) ;
#40551=EDGE_LOOP ( 'NONE', ( #45051, #27452 ) ) ;
#40552=ORIENTED_EDGE ( 'NONE', *, *, #41038, .T. ) ;
#40553=ORIENTED_EDGE ( 'NONE', *, *, #32022, .T. ) ;
#40554=CARTESIAN_POINT ( 'NONE',  ( -4.350000000000023626, 12.50000000000000000, 6.776507416713035248 ) ) ;
#40556=FACE_OUTER_BOUND ( 'NONE', #39469, .T. ) ;
#40557=CIRCLE ( 'NONE', #28013, 0.1000000000000002554 ) ;
#40558=EDGE_CURVE ( 'NONE', #41701, #87369, #45957, .T. ) ;
#40559=DIRECTION ( 'NONE',  ( -4.274815082592931898E-19, -0.9999939076577903929, -0.003490651415223739937 ) ) ;
#40560=VERTEX_POINT ( 'NONE', #49824 ) ;
#40561=CARTESIAN_POINT ( 'NONE',  ( 12.09999999999990550, 2.500000000000000000, -4.922947341949753586 ) ) ;
#40562=CARTESIAN_POINT ( 'NONE',  ( 17.37282530749035203, -0.4689596142739269613, -5.357821376857504703 ) ) ;
#40563=CARTESIAN_POINT ( 'NONE',  ( 10.84999999999990905, 2.500000000000000000, 1.472243186433545459 ) ) ;
#40564=CARTESIAN_POINT ( 'NONE',  ( -9.550000000000006040, 2.500000000000000000, 2.265063509461097357 ) ) ;
#40565=EDGE_CURVE ( 'NONE', #16136, #12100, #129038, .T. ) ;
#40566=EDGE_LOOP ( 'NONE', ( #121013, #54034 ) ) ;
#40567=DIRECTION ( 'NONE',  ( 0.000000000000000000, 1.000000000000000000, 0.000000000000000000 ) ) ;
#40568=VERTEX_POINT ( 'NONE', #10508 ) ;
#40569=ORIENTED_EDGE ( 'NONE', *, *, #28365, .T. ) ;
#40570=CARTESIAN_POINT ( 'NONE',  ( -9.400000000000007461, 2.500000000000000000, 4.776537180435972196 ) ) ;
#40571=AXIS2_PLACEMENT_3D ( 'NONE', #82354, #3774, #94089 ) ;
#40572=EDGE_CURVE ( 'NONE', #118390, #30572, #68143, .T. ) ;
#40573=CIRCLE ( 'NONE', #69791, 0.06509327318403745899 ) ;
#40574=EDGE_CURVE ( 'NONE', #46603, #6145, #119101, .T. ) ;
#40575=FACE_OUTER_BOUND ( 'NONE', #54381, .T. ) ;
#40577=FACE_BOUND ( 'NONE', #128426, .T. ) ;
#40578=EDGE_CURVE ( 'NONE', #91444, #2822, #25014, .T. ) ;
#40579=CARTESIAN_POINT ( 'NONE',  ( 12.04999999999990479, 12.50000000000000000, 2.165063509461097713 ) ) ;
#40580=CARTESIAN_POINT ( 'NONE',  ( 3.349999999999941913, 2.500000000000000000, 6.495190528383297135 ) ) ;
#40581=CARTESIAN_POINT ( 'NONE',  ( -0.2000000000000339284, 2.500000000000000000, -0.3464101615137759604 ) ) ;
#40582=CONICAL_SURFACE ( 'NONE', #124176, 0.1000000000000002554, 0.003490658503988666988 ) ;
#40583=AXIS2_PLACEMENT_3D ( 'NONE', #82720, #60504, #21865 ) ;
#40584=CONICAL_SURFACE ( 'NONE', #55230, 0.09999999999999982514, 0.003490658503988666988 ) ;
#40585=ADVANCED_FACE ( 'NONE', ( #18409 ), #98157, .T. ) ;
#40586=DIRECTION ( 'NONE',  ( 0.000000000000000000, -0.000000000000000000, 1.000000000000000000 ) ) ;
#40587=DIRECTION ( 'NONE',  ( 0.000000000000000000, 0.000000000000000000, -1.000000000000000000 ) ) ;
#40588=EDGE_CURVE ( 'NONE', #92137, #105738, #125359, .T. ) ;
#40589=CARTESIAN_POINT ( 'NONE',  ( 0.4499999999999569344, 2.500000000000000000, 2.265063509461097357 ) ) ;
#40590=DIRECTION ( 'NONE',  ( 0.000000000000000000, -0.9999939076577903929, 0.003490651415223739937 ) ) ;
#40591=ORIENTED_EDGE ( 'NONE', *, *, #46024, .T. ) ;
#40592=CONICAL_SURFACE ( 'NONE', #38530, 0.1000000000000002554, 0.003490658503988666988 ) ;
#40593=DIRECTION ( 'NONE',  ( -0.000000000000000000, -1.000000000000000000, -0.000000000000000000 ) ) ;
#40594=EDGE_CURVE ( 'NONE', #95698, #101033, #79282, .T. ) ;
#40595=AXIS2_PLACEMENT_3D ( 'NONE', #34048, #56253, #93607 ) ;
#40596=AXIS2_PLACEMENT_3D ( 'NONE', #110119, #20453, #60397 ) ;
#40597=ADVANCED_FACE ( 'NONE', ( #110653 ), #2014, .T. ) ;
#40598=DIRECTION ( 'NONE',  ( 0.000000000000000000, 0.000000000000000000, -1.000000000000000000 ) ) ;
#40599=EDGE_LOOP ( 'NONE', ( #102616, #35842 ) ) ;
#40600=ORIENTED_EDGE ( 'NONE', *, *, #64015, .T. ) ;
#40601=AXIS2_PLACEMENT_3D ( 'NONE', #118405, #16945, #78511 ) ;
#40602=DIRECTION ( 'NONE',  ( 0.000000000000000000, 0.000000000000000000, 1.000000000000000000 ) ) ;
#40603=EDGE_CURVE ( 'NONE', #20290, #61759, #4147, .T. ) ;
#40604=PLANE ( 'NONE',  #113312 ) ;
#40605=FACE_BOUND ( 'NONE', #102931, .T. ) ;
#40606=EDGE_CURVE ( 'NONE', #58961, #8339, #94061, .T. ) ;
#40607=DIRECTION ( 'NONE',  ( 0.000000000000000000, 1.000000000000000000, 0.000000000000000000 ) ) ;
#40608=DIRECTION ( 'NONE',  ( 0.000000000000000000, 0.000000000000000000, 1.000000000000000000 ) ) ;
#40609=AXIS2_PLACEMENT_3D ( 'NONE', #114340, #114973, #24682 ) ;
#40610=EDGE_LOOP ( 'NONE', ( #107998, #46626 ) ) ;
#40611=CARTESIAN_POINT ( 'NONE',  ( 8.949999999999919353, 2.500000000000000000, -6.048780366869526581 ) ) ;
#40612=CARTESIAN_POINT ( 'NONE',  ( 0.3999999999999568345, 2.500000000000000000, -5.022947341949754119 ) ) ;
#40613=AXIS2_PLACEMENT_3D ( 'NONE', #28814, #99490, #60220 ) ;
#40614=EDGE_LOOP ( 'NONE', ( #29591, #14830, #47877, #46656 ) ) ;
#40615=DIRECTION ( 'NONE',  ( -4.274815082592931898E-19, -0.9999939076577903929, -0.003490651415223739937 ) ) ;
#40616=CARTESIAN_POINT ( 'NONE',  ( -10.84999999999999964, 2.500000000000000000, 5.802370205355744659 ) ) ;
#40617=DIRECTION ( 'NONE',  ( 0.000000000000000000, 1.000000000000000000, 0.000000000000000000 ) ) ;
#40619=AXIS2_PLACEMENT_3D ( 'NONE', #13840, #4020, #45255 ) ;
#40620=VECTOR ( 'NONE', #57629, 1000.000000000000000 ) ;
#40621=ORIENTED_EDGE ( 'NONE', *, *, #4892, .F. ) ;
#40622=CARTESIAN_POINT ( 'NONE',  ( -7.700000000000010836, 12.50000000000000000, 3.983716857408420964 ) ) ;
#40623=CARTESIAN_POINT ( 'NONE',  ( 3.349999999999941913, 12.50000000000000000, 5.802370205355744659 ) ) ;
#40624=EDGE_LOOP ( 'NONE', ( #112323, #108475, #66204, #104888 ) ) ;
#40625=VERTEX_POINT ( 'NONE', #69433 ) ;
#40628=DIRECTION ( 'NONE',  ( -0.000000000000000000, -1.000000000000000000, -0.000000000000000000 ) ) ;
#40629=CARTESIAN_POINT ( 'NONE',  ( 17.50000000000000000, -2.499999999999999556, -1.333333333333328596 ) ) ;
#40630=AXIS2_PLACEMENT_3D ( 'NONE', #932, #51347, #80797 ) ;
#40631=EDGE_CURVE ( 'NONE', #106830, #106590, #20900, .T. ) ;
#40632=CARTESIAN_POINT ( 'NONE',  ( -11.05000000000000071, 2.500000000000000000, -6.741600689897074616 ) ) ;
#40633=ORIENTED_EDGE ( 'NONE', *, *, #112627, .F. ) ;
#40634=CARTESIAN_POINT ( 'NONE',  ( 1.899999999999951283, 2.500000000000000000, 0.3464101615137736845 ) ) ;
#40636=DIRECTION ( 'NONE',  ( 0.000000000000000000, 0.000000000000000000, -1.000000000000000000 ) ) ;
#40639=CARTESIAN_POINT ( 'NONE',  ( 12.29999999999990656, 2.500000000000000000, 3.883716857408421319 ) ) ;
#40640=DIRECTION ( 'NONE',  ( 0.000000000000000000, 0.000000000000000000, 1.000000000000000000 ) ) ;
#40641=EDGE_LOOP ( 'NONE', ( #127631, #47403 ) ) ;
#40642=VERTEX_POINT ( 'NONE', #38729 ) ;
#40643=DIRECTION ( 'NONE',  ( 0.000000000000000000, 1.000000000000000000, 0.000000000000000000 ) ) ;
#40644=AXIS2_PLACEMENT_3D ( 'NONE', #24941, #104763, #74043 ) ;
#40645=ORIENTED_EDGE ( 'NONE', *, *, #35527, .T. ) ;
#40646=VECTOR ( 'NONE', #71055, 1000.000000000000000 ) ;
#40647=DIRECTION ( 'NONE',  ( 0.000000000000000000, 0.000000000000000000, -1.000000000000000000 ) ) ;
#40648=ORIENTED_EDGE ( 'NONE', *, *, #102682, .F. ) ;
#40649=ORIENTED_EDGE ( 'NONE', *, *, #72373, .T. ) ;
#40651=AXIS2_PLACEMENT_3D ( 'NONE', #61028, #70214, #13203 ) ;
#40652=CARTESIAN_POINT ( 'NONE',  ( 11.04999999999991012, 2.500000000000000000, -1.818653347947326138 ) ) ;
#40653=AXIS2_PLACEMENT_3D ( 'NONE', #62631, #102532, #70497 ) ;
#40654=CARTESIAN_POINT ( 'NONE',  ( -10.65000000000000391, 2.500000000000000000, -6.048780366869523029 ) ) ;
#40655=DIRECTION ( 'NONE',  ( 0.000000000000000000, 0.000000000000000000, 1.000000000000000000 ) ) ;
#40656=DIRECTION ( 'NONE',  ( -4.274815082592931898E-19, -0.9999939076577903929, -0.003490651415223739937 ) ) ;
#40657=DIRECTION ( 'NONE',  ( 0.000000000000000000, 1.000000000000000000, 0.000000000000000000 ) ) ;
#40658=DIRECTION ( 'NONE',  ( 0.000000000000000000, 0.000000000000000000, -1.000000000000000000 ) ) ;
#40659=FACE_OUTER_BOUND ( 'NONE', #37690, .T. ) ;
#40660=DIRECTION ( 'NONE',  ( 0.000000000000000000, 0.000000000000000000, 1.000000000000000000 ) ) ;
#40661=LINE ( 'NONE', #13082, #8000 ) ;
#40662=ORIENTED_EDGE ( 'NONE', *, *, #114950, .F. ) ;
#40663=AXIS2_PLACEMENT_3D ( 'NONE', #54186, #12942, #14236 ) ;
#40664=CARTESIAN_POINT ( 'NONE',  ( 9.349999999999919709, 12.50000000000000000, -6.776507416713040577 ) ) ;
#40665=AXIS2_PLACEMENT_3D ( 'NONE', #120815, #31167, #2980 ) ;
#40666=AXIS2_PLACEMENT_3D ( 'NONE', #93408, #4347, #104506 ) ;
#40668=ORIENTED_EDGE ( 'NONE', *, *, #50079, .T. ) ;
#40669=LINE ( 'NONE', #70747, #81669 ) ;
#40670=DIRECTION ( 'NONE',  ( 0.000000000000000000, -0.000000000000000000, 1.000000000000000000 ) ) ;
#40671=ADVANCED_FACE ( 'NONE', ( #39368 ), #35492, .T. ) ;
#40672=CIRCLE ( 'NONE', #124175, 0.1000000000000002554 ) ;
#40673=VECTOR ( 'NONE', #42419, 1000.000000000000000 ) ;
#40675=AXIS2_PLACEMENT_3D ( 'NONE', #84091, #124684, #106324 ) ;
#40676=CARTESIAN_POINT ( 'NONE',  ( -1.650000000000034328, 2.500000000000000000, -7.088010851410853519 ) ) ;
#40677=DIRECTION ( 'NONE',  ( 0.000000000000000000, -0.9999939076577903929, 0.003490651415223739937 ) ) ;
#40678=PLANE ( 'NONE',  #126245 ) ;
#40679=VERTEX_POINT ( 'NONE', #59661 ) ;
#40680=AXIS2_PLACEMENT_3D ( 'NONE', #62075, #102619, #11668 ) ;
#40681=EDGE_LOOP ( 'NONE', ( #123758, #34023, #86395, #120343 ) ) ;
#40682=CARTESIAN_POINT ( 'NONE',  ( -0.4000000000000396572, 12.50000000000000000, 3.702399969078682407 ) ) ;
#40683=VECTOR ( 'NONE', #35287, 1000.000000000000000 ) ;
#40684=ORIENTED_EDGE ( 'NONE', *, *, #74829, .F. ) ;
#40685=DIRECTION ( 'NONE',  ( 0.000000000000000000, 0.000000000000000000, 1.000000000000000000 ) ) ;
#40686=ORIENTED_EDGE ( 'NONE', *, *, #105840, .F. ) ;
#40687=AXIS2_PLACEMENT_3D ( 'NONE', #6986, #127443, #25346 ) ;
#40688=EDGE_CURVE ( 'NONE', #69752, #18590, #91910, .T. ) ;
#40689=EDGE_CURVE ( 'NONE', #105649, #115836, #92475, .T. ) ;
#40690=ORIENTED_EDGE ( 'NONE', *, *, #11883, .T. ) ;
#40691=CARTESIAN_POINT ( 'NONE',  ( 4.599999999999937472, 12.50000000000000000, 0.7579135962115869374 ) ) ;
#40692=DIRECTION ( 'NONE',  ( -0.000000000000000000, 1.000000000000000000, -0.000000000000000000 ) ) ;
#40693=CARTESIAN_POINT ( 'NONE',  ( -3.550000000000027800, 2.500000000000000000, 6.148780366869520009 ) ) ;
#40694=DIRECTION ( 'NONE',  ( 0.000000000000000000, -0.000000000000000000, 1.000000000000000000 ) ) ;
#40695=CARTESIAN_POINT ( 'NONE',  ( 87.50000000000002842, 0.7169905660283034665, 7.500000000000000888 ) ) ;
#40697=DIRECTION ( 'NONE',  ( 0.000000000000000000, 0.000000000000000000, 1.000000000000000000 ) ) ;
#40698=CARTESIAN_POINT ( 'NONE',  ( 3.349999999999944578, 2.500000000000000000, -1.472243186433550122 ) ) ;
#40699=EDGE_CURVE ( 'NONE', #102274, #88216, #98898, .T. ) ;
#40700=CARTESIAN_POINT ( 'NONE',  ( -10.85000000000000142, 2.500000000000000000, -7.188010851410850499 ) ) ;
#40701=CARTESIAN_POINT ( 'NONE',  ( 7.699999999999923794, 2.500000000000000000, -4.083716857408426826 ) ) ;
#40702=VECTOR ( 'NONE', #3470, 1000.000000000000000 ) ;
#40703=CARTESIAN_POINT ( 'NONE',  ( 6.049999999999932321, 2.500000000000000000, 6.941600689897073018 ) ) ;
#40704=ORIENTED_EDGE ( 'NONE', *, *, #78020, .T. ) ;
#40705=ORIENTED_EDGE ( 'NONE', *, *, #26984, .F. ) ;
#40706=CARTESIAN_POINT ( 'NONE',  ( 6.899999999999926636, 12.50000000000000000, 0.3464101615137736845 ) ) ;
#40707=ORIENTED_EDGE ( 'NONE', *, *, #75288, .T. ) ;
#40708=CONICAL_SURFACE ( 'NONE', #53219, 0.1000000000000002554, 0.003490658503988666988 ) ;
#40709=DIRECTION ( 'NONE',  ( -4.274815082592931898E-19, -0.9999939076577903929, -0.003490651415223739937 ) ) ;
#40710=DIRECTION ( 'NONE',  ( 0.000000000000000000, 0.000000000000000000, -1.000000000000000000 ) ) ;
#40711=AXIS2_PLACEMENT_3D ( 'NONE', #18331, #9165, #109954 ) ;
#40712=EDGE_LOOP ( 'NONE', ( #13464, #52779, #17929, #49239 ) ) ;
#40713=FACE_OUTER_BOUND ( 'NONE', #14932, .T. ) ;
#40714=CARTESIAN_POINT ( 'NONE',  ( 8.349999999999923261, 2.500000000000000000, 1.472243186433545459 ) ) ;
#40715=CARTESIAN_POINT ( 'NONE',  ( -2.300000000000033573, 2.500000000000000000, 4.676537180435972552 ) ) ;
#40716=CARTESIAN_POINT ( 'NONE',  ( -6.505213034913026604E-15, 12.50000000000000000, 4.395220292106234439 ) ) ;
#40717=AXIS2_PLACEMENT_3D ( 'NONE', #26383, #36205, #16527 ) ;
#40718=EDGE_CURVE ( 'NONE', #108142, #90854, #15181, .T. ) ;
#40719=DIRECTION ( 'NONE',  ( -0.000000000000000000, -1.000000000000000000, -0.000000000000000000 ) ) ;
#40720=CIRCLE ( 'NONE', #11536, 0.06509327318403745899 ) ;
#40721=EDGE_LOOP ( 'NONE', ( #88327, #116338, #65051, #99708 ) ) ;
#40722=EDGE_CURVE ( 'NONE', #52069, #1010, #112601, .T. ) ;
#40723=CARTESIAN_POINT ( 'NONE',  ( 3.549999999999942091, 2.500000000000000000, 2.611473670974873151 ) ) ;
#40724=DIRECTION ( 'NONE',  ( 0.000000000000000000, -0.000000000000000000, 1.000000000000000000 ) ) ;
#40725=EDGE_CURVE ( 'NONE', #8118, #21551, #14370, .T. ) ;
#40726=CARTESIAN_POINT ( 'NONE',  ( -12.09999999999999609, 2.500000000000000000, 1.734723475976807094E-15 ) ) ;
#40727=DIRECTION ( 'NONE',  ( 0.000000000000000000, 0.000000000000000000, 1.000000000000000000 ) ) ;
#40728=VERTEX_POINT ( 'NONE', #73957 ) ;
#40729=AXIS2_PLACEMENT_3D ( 'NONE', #6271, #76329, #104489 ) ;
#40730=ADVANCED_FACE ( 'NONE', ( #83773 ), #53033, .T. ) ;
#40731=EDGE_CURVE ( 'NONE', #124558, #128215, #27715, .T. ) ;
#40732=CIRCLE ( 'NONE', #73874, 0.06509327318403745899 ) ;
#40733=VERTEX_POINT ( 'NONE', #54317 ) ;
#40734=DIRECTION ( 'NONE',  ( -0.000000000000000000, -1.000000000000000000, -0.000000000000000000 ) ) ;
#40735=CARTESIAN_POINT ( 'NONE',  ( -13.54999999999998828, 2.500000000000000000, 1.918653347947325338 ) ) ;
#40736=EDGE_CURVE ( 'NONE', #43212, #24381, #4369, .T. ) ;
#40737=CARTESIAN_POINT ( 'NONE',  ( -9.600000000000006750, 12.50000000000000000, 0.6928203230275494784 ) ) ;
#40738=AXIS2_PLACEMENT_3D ( 'NONE', #57957, #79527, #18665 ) ;
#40739=ORIENTED_EDGE ( 'NONE', *, *, #107150, .T. ) ;
#40740=CARTESIAN_POINT ( 'NONE',  ( -2.050000000000033129, 12.50000000000000000, 6.495190528383297135 ) ) ;
#40741=ADVANCED_FACE ( 'NONE', ( #93595 ), #48572, .T. ) ;
#40742=DIRECTION ( 'NONE',  ( 0.000000000000000000, 0.000000000000000000, 1.000000000000000000 ) ) ;
#40743=ORIENTED_EDGE ( 'NONE', *, *, #19703, .T. ) ;
#40744=PLANE ( 'NONE',  #97049 ) ;
#40745=ORIENTED_EDGE ( 'NONE', *, *, #108875, .T. ) ;
#40746=ADVANCED_FACE ( 'NONE', ( #72674 ), #62848, .T. ) ;
#40747=DIRECTION ( 'NONE',  ( -1.000000000000000000, 0.000000000000000000, 0.000000000000000000 ) ) ;
#40748=AXIS2_PLACEMENT_3D ( 'NONE', #40518, #41808, #88955 ) ;
#40749=VERTEX_POINT ( 'NONE', #2619 ) ;
#40751=CARTESIAN_POINT ( 'NONE',  ( 7.173569985920779324, 2.499999999999999112, -8.713264184442468974 ) ) ;
#40752=CONICAL_SURFACE ( 'NONE', #92969, 0.1000000000000000472, 0.003490658503988666988 ) ;
#40753=AXIS2_PLACEMENT_3D ( 'NONE', #17947, #117407, #108258 ) ;
#40754=ORIENTED_EDGE ( 'NONE', *, *, #60099, .T. ) ;
#40755=ORIENTED_EDGE ( 'NONE', *, *, #20196, .F. ) ;
#40756=LINE ( 'NONE', #112054, #114586 ) ;
#40757=CARTESIAN_POINT ( 'NONE',  ( -0.6500000000000394351, 12.50000000000000000, 2.576566944158910744 ) ) ;
#40758=ORIENTED_EDGE ( 'NONE', *, *, #31960, .T. ) ;
#40759=FACE_OUTER_BOUND ( 'NONE', #59799, .T. ) ;
#40760=CARTESIAN_POINT ( 'NONE',  ( 1.849999999999949685, 2.500000000000000000, -2.411473670974877859 ) ) ;
#40761=AXIS2_PLACEMENT_3D ( 'NONE', #12919, #127414, #64617 ) ;
#40762=CONICAL_SURFACE ( 'NONE', #76255, 0.1000000000000000472, 0.003490658503988666988 ) ;
#40763=CARTESIAN_POINT ( 'NONE',  ( 13.29999999999990301, 12.50000000000000000, 4.395220292106234439 ) ) ;
#40765=DIRECTION ( 'NONE',  ( 0.000000000000000000, 1.000000000000000000, 0.000000000000000000 ) ) ;
#40766=AXIS2_PLACEMENT_3D ( 'NONE', #19411, #60658, #100559 ) ;
#40767=DIRECTION ( 'NONE',  ( 0.000000000000000000, 0.000000000000000000, 1.000000000000000000 ) ) ;
#40769=CIRCLE ( 'NONE', #90920, 0.06509327318403745899 ) ;
#40770=VECTOR ( 'NONE', #91297, 1000.000000000000000 ) ;
#40771=EDGE_LOOP ( 'NONE', ( #121724, #20163, #53519, #78912 ) ) ;
#40772=EDGE_LOOP ( 'NONE', ( #8204, #116627 ) ) ;
#40773=ORIENTED_EDGE ( 'NONE', *, *, #25263, .T. ) ;
#40774=FACE_OUTER_BOUND ( 'NONE', #13488, .T. ) ;
#40775=DIRECTION ( 'NONE',  ( -4.274815082592931898E-19, -0.9999939076577903929, -0.003490651415223739937 ) ) ;
#40776=AXIS2_PLACEMENT_3D ( 'NONE', #35202, #75114, #102625 ) ;
#40777=DIRECTION ( 'NONE',  ( 0.000000000000000000, 0.000000000000000000, 1.000000000000000000 ) ) ;
#40778=ORIENTED_EDGE ( 'NONE', *, *, #80020, .F. ) ;
#40779=ORIENTED_EDGE ( 'NONE', *, *, #84425, .T. ) ;
#40780=FACE_BOUND ( 'NONE', #7269, .T. ) ;
#40781=EDGE_LOOP ( 'NONE', ( #119177, #80715 ) ) ;
#40782=DIRECTION ( 'NONE',  ( 0.000000000000000000, 0.000000000000000000, 1.000000000000000000 ) ) ;
#40783=CARTESIAN_POINT ( 'NONE',  ( -6.850000000000013856, 2.500000000000000000, 2.511473670974873507 ) ) ;
#40784=CARTESIAN_POINT ( 'NONE',  ( -9.400000000000007461, 2.500000000000000000, 0.2464101615137735679 ) ) ;
#40785=CARTESIAN_POINT ( 'NONE',  ( 8.549999999999922551, 2.500000000000000000, -6.048780366869526581 ) ) ;
#40788=CARTESIAN_POINT ( 'NONE',  ( -3.150000000000030553, 12.50000000000000000, 6.083687093685482772 ) ) ;
#40789=DIRECTION ( 'NONE',  ( 0.000000000000000000, -0.9999939076577903929, 0.003490651415223739937 ) ) ;
#40790=DIRECTION ( 'NONE',  ( 0.000000000000000000, 0.000000000000000000, -1.000000000000000000 ) ) ;
#40791=CARTESIAN_POINT ( 'NONE',  ( -4.600000000000025402, 2.500000000000000000, 0.09999999999999761857 ) ) ;
#40792=AXIS2_PLACEMENT_3D ( 'NONE', #59108, #31577, #9356 ) ;
#40793=DIRECTION ( 'NONE',  ( -0.000000000000000000, -1.000000000000000000, -0.000000000000000000 ) ) ;
#40794=EDGE_CURVE ( 'NONE', #60983, #7100, #23510, .T. ) ;
#40795=ORIENTED_EDGE ( 'NONE', *, *, #68890, .T. ) ;
#40796=VERTEX_POINT ( 'NONE', #1982 ) ;
#40797=ORIENTED_EDGE ( 'NONE', *, *, #74240, .T. ) ;
#40798=EDGE_LOOP ( 'NONE', ( #86681, #73798 ) ) ;
#40799=CARTESIAN_POINT ( 'NONE',  ( -12.89999999999999147, 2.500000000000000000, -5.022947341949751454 ) ) ;
#40800=DIRECTION ( 'NONE',  ( -4.274815082592931898E-19, -0.9999939076577903929, -0.003490651415223739937 ) ) ;
#40801=ORIENTED_EDGE ( 'NONE', *, *, #7628, .F. ) ;
#40802=EDGE_LOOP ( 'NONE', ( #89229, #126062, #29632, #67122 ) ) ;
#40803=ORIENTED_EDGE ( 'NONE', *, *, #128005, .F. ) ;
#40804=DIRECTION ( 'NONE',  ( 0.000000000000000000, -0.9999939076577903929, 0.003490651415223739937 ) ) ;
#40805=AXIS2_PLACEMENT_3D ( 'NONE', #67925, #99334, #70502 ) ;
#40806=CARTESIAN_POINT ( 'NONE',  ( -3.469446951953614189E-14, 12.50000000000000000, -0.6928203230275519209 ) ) ;
#40807=( NAMED_UNIT ( * ) PLANE_ANGLE_UNIT ( ) SI_UNIT ( $, .RADIAN. ) );
#40808=DIRECTION ( 'NONE',  ( -0.000000000000000000, 1.000000000000000000, -0.000000000000000000 ) ) ;
#40809=DIRECTION ( 'NONE',  ( 0.000000000000000000, 0.000000000000000000, 1.000000000000000000 ) ) ;
#40810=DIRECTION ( 'NONE',  ( 0.000000000000000000, 1.000000000000000000, 0.000000000000000000 ) ) ;
#40811=DIRECTION ( 'NONE',  ( 0.000000000000000000, 0.000000000000000000, 1.000000000000000000 ) ) ;
#40812=ORIENTED_EDGE ( 'NONE', *, *, #109896, .T. ) ;
#40813=DIRECTION ( 'NONE',  ( 0.000000000000000000, 0.000000000000000000, 1.000000000000000000 ) ) ;
#40814=VERTEX_POINT ( 'NONE', #111276 ) ;
#40815=AXIS2_PLACEMENT_3D ( 'NONE', #62918, #53106, #64197 ) ;
#40816=ORIENTED_EDGE ( 'NONE', *, *, #15056, .T. ) ;
#40817=VERTEX_POINT ( 'NONE', #121120 ) ;
#40818=VECTOR ( 'NONE', #37219, 1000.000000000000000 ) ;
#40819=CARTESIAN_POINT ( 'NONE',  ( 3.749999999999978684, 2.500000000000000000, -6.495190528383302464 ) ) ;
#40820=ORIENTED_EDGE ( 'NONE', *, *, #50809, .T. ) ;
#40821=EDGE_LOOP ( 'NONE', ( #84318, #29981, #95771, #55611 ) ) ;
#40822=VERTEX_POINT ( 'NONE', #61577 ) ;
#40823=CARTESIAN_POINT ( 'NONE',  ( -4.550000000000022915, 12.50000000000000000, -2.165063509461101710 ) ) ;
#40824=ADVANCED_FACE ( 'NONE', ( #33407 ), #40254, .T. ) ;
#40825=CARTESIAN_POINT ( 'NONE',  ( -8.350000000000013856, 2.500000000000000000, -6.495190528383297135 ) ) ;
#40826=AXIS2_PLACEMENT_3D ( 'NONE', #61836, #102395, #53933 ) ;
#40827=CARTESIAN_POINT ( 'NONE',  ( 6.649999999999928413, 12.50000000000000000, 2.857883832488649301 ) ) ;
#40828=CONICAL_SURFACE ( 'NONE', #24083, 0.1000000000000002554, 0.003490658503988666988 ) ;
#40829=DIRECTION ( 'NONE',  ( -0.000000000000000000, 1.000000000000000000, -0.000000000000000000 ) ) ;
#40830=CARTESIAN_POINT ( 'NONE',  ( -3.300000000000027800, 12.50000000000000000, -2.276824562219559311E-15 ) ) ;
#40831=CARTESIAN_POINT ( 'NONE',  ( -1.050000000000038680, 12.50000000000000000, 6.841600689897072485 ) ) ;
#40832=CARTESIAN_POINT ( 'NONE',  ( -3.300000000000028244, 12.50000000000000000, 4.265033745738159077 ) ) ;
#40833=EDGE_CURVE ( 'NONE', #127817, #77958, #81830, .T. ) ;
#40834=ORIENTED_EDGE ( 'NONE', *, *, #73839, .T. ) ;
#40835=FACE_OUTER_BOUND ( 'NONE', #106260, .T. ) ;
#40836=EDGE_LOOP ( 'NONE', ( #120826, #14178, #49371, #21860 ) ) ;
#40838=DIRECTION ( 'NONE',  ( 0.000000000000000000, 1.000000000000000000, 0.000000000000000000 ) ) ;
#40839=VERTEX_POINT ( 'NONE', #11806 ) ;
#40840=CARTESIAN_POINT ( 'NONE',  ( -5.850000000000021849, 2.500000000000000000, -1.372243186433550033 ) ) ;
#40842=DIRECTION ( 'NONE',  ( 0.000000000000000000, 1.000000000000000000, 0.000000000000000000 ) ) ;
#40843=ADVANCED_FACE ( 'NONE', ( #63496 ), #122423, .T. ) ;
#40844=CIRCLE ( 'NONE', #118174, 0.06509327318403745899 ) ;
#40845=ORIENTED_EDGE ( 'NONE', *, *, #122133, .F. ) ;
#40846=CONICAL_SURFACE ( 'NONE', #103514, 0.09999999999999999167, 0.003490658503988666988 ) ;
#40847=EDGE_CURVE ( 'NONE', #51297, #63587, #121757, .T. ) ;
#40848=VECTOR ( 'NONE', #57248, 1000.000000000000000 ) ;
#40849=CARTESIAN_POINT ( 'NONE',  ( -0.2000000000000412836, 12.50000000000000000, 4.611443907251934426 ) ) ;
#40850=ORIENTED_EDGE ( 'NONE', *, *, #31383, .T. ) ;
#40851=CIRCLE ( 'NONE', #118181, 0.09999999999999999167 ) ;
#40852=VERTEX_POINT ( 'NONE', #17598 ) ;
#40853=DIRECTION ( 'NONE',  ( 0.000000000000000000, 0.000000000000000000, 1.000000000000000000 ) ) ;
#40854=CARTESIAN_POINT ( 'NONE',  ( -9.200000000000009948, 2.500000000000000000, -4.330127018922197202 ) ) ;
#40855=ADVANCED_FACE ( 'NONE', ( #34700 ), #104687, .T. ) ;
#40857=CARTESIAN_POINT ( 'NONE',  ( -13.94999999999998685, 2.500000000000000000, -2.611473670974875372 ) ) ;
#40858=CIRCLE ( 'NONE', #32536, 0.1000000000000002554 ) ;
#40859=DIRECTION ( 'NONE',  ( 0.000000000000000000, 1.000000000000000000, 0.000000000000000000 ) ) ;
#40860=CIRCLE ( 'NONE', #70078, 0.09999999999999982514 ) ;
#40861=ORIENTED_EDGE ( 'NONE', *, *, #61831, .T. ) ;
#40862=AXIS2_PLACEMENT_3D ( 'NONE', #97636, #111141, #50974 ) ;
#40863=DIRECTION ( 'NONE',  ( 0.000000000000000000, 1.000000000000000000, 0.000000000000000000 ) ) ;
#40864=VECTOR ( 'NONE', #84790, 1000.000000000000000 ) ;
#40865=ORIENTED_EDGE ( 'NONE', *, *, #39432, .T. ) ;
#40866=CONICAL_SURFACE ( 'NONE', #42924, 0.09999999999999982514, 0.003490658503988666988 ) ;
#40867=CARTESIAN_POINT ( 'NONE',  ( -5.450000000000023270, 12.50000000000000000, -2.165063509461101710 ) ) ;
#40868=CARTESIAN_POINT ( 'NONE',  ( -8.550000000000013145, 2.500000000000000000, -6.841600689897073373 ) ) ;
#40869=CONICAL_SURFACE ( 'NONE', #99438, 0.1000000000000002554, 0.003490658503988666988 ) ;
#40870=ADVANCED_FACE ( 'NONE', ( #15656 ), #96660, .T. ) ;
#40871=AXIS2_PLACEMENT_3D ( 'NONE', #97651, #116642, #108750 ) ;
#40873=CARTESIAN_POINT ( 'NONE',  ( 11.04999999999990656, 2.500000000000000000, 2.511473670974873507 ) ) ;
#40874=DIRECTION ( 'NONE',  ( 0.000000000000000000, 1.000000000000000000, 0.000000000000000000 ) ) ;
#40875=CARTESIAN_POINT ( 'NONE',  ( 1.249999999999952482, 12.50000000000000000, -5.737276932171712751 ) ) ;
#40876=CARTESIAN_POINT ( 'NONE',  ( -9.150000000000005684, 12.50000000000000000, 6.560283801567334372 ) ) ;
#40877=VERTEX_POINT ( 'NONE', #117082 ) ;
#40878=DIRECTION ( 'NONE',  ( 0.000000000000000000, 0.000000000000000000, -1.000000000000000000 ) ) ;
#40879=EDGE_CURVE ( 'NONE', #82797, #7894, #107132, .T. ) ;
#40880=CARTESIAN_POINT ( 'NONE',  ( 6.449999999999931788, 2.500000000000000000, 6.048780366869520364 ) ) ;
#40881=DIRECTION ( 'NONE',  ( 0.000000000000000000, 0.000000000000000000, -1.000000000000000000 ) ) ;
#40882=AXIS2_PLACEMENT_3D ( 'NONE', #48479, #129003, #60256 ) ;
#40883=ORIENTED_EDGE ( 'NONE', *, *, #28024, .F. ) ;
#40885=DIRECTION ( 'NONE',  ( -0.000000000000000000, 1.000000000000000000, -0.000000000000000000 ) ) ;
#40886=ORIENTED_EDGE ( 'NONE', *, *, #29123, .F. ) ;
#40887=B_SPLINE_SURFACE_WITH_KNOTS ( 'NONE', 3, 1, ( 
 ( #21020, #41333 ),
 ( #81863, #90 ),
 ( #91055, #1373 ),
 ( #32802, #22966 ),
 ( #99599, #79942 ),
 ( #40695, #119868 ),
 ( #20388, #70770 ),
 ( #60330, #50484 ),
 ( #90391, #730 ),
 ( #73995, #104722 ) ),
 .UNSPECIFIED., .F., .F., .F.,
 ( 4, 2, 2, 2, 4 ),
 ( 2, 2 ),
 ( 0.000000000000000000, 0.2499999999999999445, 0.4999999999999998890, 0.7499999999999998890, 1.000000000000000000 ),
 ( 0.000000000000000000, 1.000000000000000000 ),
 .UNSPECIFIED. ) ;
#40888=ORIENTED_EDGE ( 'NONE', *, *, #105533, .T. ) ;
#40889=FACE_OUTER_BOUND ( 'NONE', #105247, .T. ) ;
#40891=AXIS2_PLACEMENT_3D ( 'NONE', #12567, #30952, #51242 ) ;
#40892=ORIENTED_EDGE ( 'NONE', *, *, #88119, .T. ) ;
#40893=DIRECTION ( 'NONE',  ( 0.000000000000000000, 0.000000000000000000, 1.000000000000000000 ) ) ;
#40894=DIRECTION ( 'NONE',  ( 0.000000000000000000, 0.000000000000000000, -1.000000000000000000 ) ) ;
#40895=EDGE_CURVE ( 'NONE', #104198, #77609, #24856, .T. ) ;
#40896=EDGE_CURVE ( 'NONE', #76783, #70057, #6462, .T. ) ;
#40897=AXIS2_PLACEMENT_3D ( 'NONE', #27198, #125408, #84181 ) ;
#40898=ORIENTED_EDGE ( 'NONE', *, *, #1637, .T. ) ;
#40899=CARTESIAN_POINT ( 'NONE',  ( -9.350000000000004974, 2.500000000000000000, 6.248780366869521430 ) ) ;
#40900=ADVANCED_FACE ( 'NONE', ( #46417 ), #6763, .T. ) ;
#40901=DIRECTION ( 'NONE',  ( 0.000000000000000000, 1.000000000000000000, 0.000000000000000000 ) ) ;
#40902=CARTESIAN_POINT ( 'NONE',  ( 4.149999999999938183, 2.500000000000000000, 5.802370205355744659 ) ) ;
#40903=ORIENTED_EDGE ( 'NONE', *, *, #77093, .F. ) ;
#40904=EDGE_CURVE ( 'NONE', #46019, #94540, #67397, .T. ) ;
#40905=VECTOR ( 'NONE', #86410, 1000.000000000000000 ) ;
#40906=ADVANCED_FACE ( 'NONE', ( #125615 ), #117580, .T. ) ;
#40907=VERTEX_POINT ( 'NONE', #37267 ) ;
#40908=CIRCLE ( 'NONE', #114049, 0.09999999999999982514 ) ;
#40910=CARTESIAN_POINT ( 'NONE',  ( -14.54999999999998472, 12.50000000000000000, 2.165063509461101265 ) ) ;
#40911=DIRECTION ( 'NONE',  ( 0.000000000000000000, -0.9999939076577903929, 0.003490651415223739937 ) ) ;
#40912=CARTESIAN_POINT ( 'NONE',  ( 9.399999999999918643, 2.500000000000000000, -0.2464101615137782308 ) ) ;
#40913=FACE_BOUND ( 'NONE', #58776, .T. ) ;
#40914=ORIENTED_EDGE ( 'NONE', *, *, #85480, .T. ) ;
#40915=CARTESIAN_POINT ( 'NONE',  ( -0.8500000000000382805, 2.500000000000000000, -7.288010851410854585 ) ) ;
#40916=CARTESIAN_POINT ( 'NONE',  ( 3.549999999999943867, 2.500000000000000000, -6.248780366869526759 ) ) ;
#40917=ORIENTED_EDGE ( 'NONE', *, *, #807, .F. ) ;
#40918=DIRECTION ( 'NONE',  ( -0.000000000000000000, 1.000000000000000000, -0.000000000000000000 ) ) ;
#40919=AXIS2_PLACEMENT_3D ( 'NONE', #111558, #21910, #63759 ) ;
#40920=DIRECTION ( 'NONE',  ( 0.000000000000000000, 1.000000000000000000, 0.000000000000000000 ) ) ;
#40921=AXIS2_PLACEMENT_3D ( 'NONE', #86628, #55251, #63785 ) ;
#40922=DIRECTION ( 'NONE',  ( -0.000000000000000000, 1.000000000000000000, -0.000000000000000000 ) ) ;
#40923=DIRECTION ( 'NONE',  ( -0.000000000000000000, -1.000000000000000000, -0.000000000000000000 ) ) ;
#40924=DIRECTION ( 'NONE',  ( 0.000000000000000000, 0.000000000000000000, 1.000000000000000000 ) ) ;
#40925=CARTESIAN_POINT ( 'NONE',  ( -6.900000000000015454, 2.500000000000000000, 4.576537180435972019 ) ) ;
#40926=ADVANCED_FACE ( 'NONE', ( #35330 ), #61177, .T. ) ;
#40927=CARTESIAN_POINT ( 'NONE',  ( 9.199999999999919353, 2.500000000000000000, 0.09999999999999772959 ) ) ;
#40929=ORIENTED_EDGE ( 'NONE', *, *, #29024, .T. ) ;
#40930=EDGE_LOOP ( 'NONE', ( #70665, #120877 ) ) ;
#40931=ORIENTED_EDGE ( 'NONE', *, *, #110876, .T. ) ;
#40932=DIRECTION ( 'NONE',  ( 0.000000000000000000, 1.000000000000000000, 0.000000000000000000 ) ) ;
#40933=CARTESIAN_POINT ( 'NONE',  ( 5.649999999999932854, 2.500000000000000000, 2.511473670974873507 ) ) ;
#40934=ORIENTED_EDGE ( 'NONE', *, *, #104995, .F. ) ;
#40935=FACE_BOUND ( 'NONE', #54357, .T. ) ;
#40936=AXIS2_PLACEMENT_3D ( 'NONE', #71219, #120968, #41144 ) ;
#40937=DIRECTION ( 'NONE',  ( -0.000000000000000000, 1.000000000000000000, -0.000000000000000000 ) ) ;
#40938=CARTESIAN_POINT ( 'NONE',  ( 6.649999999999930189, 2.500000000000000000, -1.472243186433550122 ) ) ;
#40939=AXIS2_PLACEMENT_3D ( 'NONE', #62354, #61712, #82638 ) ;
#40940=CARTESIAN_POINT ( 'NONE',  ( 8.549999999999920774, 2.500000000000000000, 6.048780366869521252 ) ) ;
#40941=VECTOR ( 'NONE', #901, 1000.000000000000000 ) ;
#40942=FACE_OUTER_BOUND ( 'NONE', #107084, .T. ) ;
#40943=CARTESIAN_POINT ( 'NONE',  ( 4.599999999999939249, 12.50000000000000000, -3.572213422710612374 ) ) ;
#40944=DIRECTION ( 'NONE',  ( -0.000000000000000000, -1.000000000000000000, -0.000000000000000000 ) ) ;
#40945=FACE_OUTER_BOUND ( 'NONE', #83496, .T. ) ;
#40946=LINE ( 'NONE', #23199, #74786 ) ;
#40947=ORIENTED_EDGE ( 'NONE', *, *, #40904, .F. ) ;
#40948=AXIS2_PLACEMENT_3D ( 'NONE', #12465, #24233, #125007 ) ;
#40949=EDGE_LOOP ( 'NONE', ( #117562, #60051, #86869, #42468 ) ) ;
#40950=EDGE_CURVE ( 'NONE', #84951, #124476, #31841, .T. ) ;
#40951=VERTEX_POINT ( 'NONE', #96802 ) ;
#40952=VERTEX_POINT ( 'NONE', #67321 ) ;
#40953=ORIENTED_EDGE ( 'NONE', *, *, #19572, .T. ) ;
#40954=VERTEX_POINT ( 'NONE', #85057 ) ;
#40955=AXIS2_PLACEMENT_3D ( 'NONE', #110236, #120701, #28466 ) ;
#40956=CARTESIAN_POINT ( 'NONE',  ( -11.64999999999999680, 2.500000000000000000, 2.165063509461097713 ) ) ;
#40957=EDGE_LOOP ( 'NONE', ( #108599, #24528, #25369, #92464 ) ) ;
#40958=CIRCLE ( 'NONE', #99437, 0.1000000000000002554 ) ;
#40959=AXIS2_PLACEMENT_3D ( 'NONE', #76662, #45923, #87115 ) ;
#40960=CONICAL_SURFACE ( 'NONE', #84757, 0.09999999999999982514, 0.003490658503988666988 ) ;
#40961=CARTESIAN_POINT ( 'NONE',  ( 19.52519901027826421, 0.5909487300084502737, 4.333354523369964184 ) ) ;
#40963=DIRECTION ( 'NONE',  ( 0.000000000000000000, 1.000000000000000000, 0.000000000000000000 ) ) ;
#40964=CARTESIAN_POINT ( 'NONE',  ( 4.399999999999939071, 12.50000000000000000, 0.3464101615137736845 ) ) ;
#40965=VECTOR ( 'NONE', #111995, 1000.000000000000000 ) ;
#40966=ORIENTED_EDGE ( 'NONE', *, *, #36751, .F. ) ;
#40967=DIRECTION ( 'NONE',  ( 0.000000000000000000, -0.000000000000000000, 1.000000000000000000 ) ) ;
#40968=EDGE_LOOP ( 'NONE', ( #97896, #7811 ) ) ;
#40969=ORIENTED_EDGE ( 'NONE', *, *, #20634, .T. ) ;
#40970=FACE_OUTER_BOUND ( 'NONE', #8662, .T. ) ;
#40971=FACE_OUTER_BOUND ( 'NONE', #2919, .T. ) ;
#40972=DIRECTION ( 'NONE',  ( 0.000000000000000000, 0.000000000000000000, 1.000000000000000000 ) ) ;
#40973=CIRCLE ( 'NONE', #74396, 0.1000000000000000472 ) ;
#40974=EDGE_LOOP ( 'NONE', ( #19576, #117685, #42363, #70440 ) ) ;
#40975=ORIENTED_EDGE ( 'NONE', *, *, #50834, .T. ) ;
#40976=CARTESIAN_POINT ( 'NONE',  ( 11.64999999999990798, 2.500000000000000000, -1.472243186433550122 ) ) ;
#40977=DIRECTION ( 'NONE',  ( 0.000000000000000000, 0.000000000000000000, -1.000000000000000000 ) ) ;
#40978=DIRECTION ( 'NONE',  ( 0.000000000000000000, 0.000000000000000000, -1.000000000000000000 ) ) ;
#40979=CARTESIAN_POINT ( 'NONE',  ( 10.44999999999991047, 2.500000000000000000, -6.395190528383301931 ) ) ;
#40980=ORIENTED_EDGE ( 'NONE', *, *, #113086, .T. ) ;
#40981=DIRECTION ( 'NONE',  ( 0.000000000000000000, -0.9999939076577903929, 0.003490651415223739937 ) ) ;
#40982=CIRCLE ( 'NONE', #93195, 0.09999999999999999167 ) ;
#40983=ORIENTED_EDGE ( 'NONE', *, *, #42807, .F. ) ;
#40984=DIRECTION ( 'NONE',  ( 0.000000000000000000, -0.9999939076577903929, 0.003490651415223739937 ) ) ;
#40985=AXIS2_PLACEMENT_3D ( 'NONE', #12701, #92573, #82773 ) ;
#40986=ADVANCED_FACE ( 'NONE', ( #107278 ), #42308, .T. ) ;
#40987=VERTEX_POINT ( 'NONE', #84416 ) ;
#40989=CARTESIAN_POINT ( 'NONE',  ( -3.100000000000028511, 2.500000000000000000, -3.983716857408426293 ) ) ;
#40990=CARTESIAN_POINT ( 'NONE',  ( 6.849999999999929479, 2.500000000000000000, 6.248780366869520542 ) ) ;
#40991=LINE ( 'NONE', #2308, #28125 ) ;
#40992=EDGE_CURVE ( 'NONE', #90531, #41827, #77883, .T. ) ;
#40993=CARTESIAN_POINT ( 'NONE',  ( -9.600000000000008527, 12.50000000000000000, -4.330127018922197202 ) ) ;
#40994=EDGE_CURVE ( 'NONE', #13065, #85675, #45155, .T. ) ;
#40995=VERTEX_POINT ( 'NONE', #75239 ) ;
#40996=CIRCLE ( 'NONE', #43146, 0.06509327318403745899 ) ;
#40997=CARTESIAN_POINT ( 'NONE',  ( -9.150000000000009237, 2.500000000000000000, -2.757883832488654097 ) ) ;
#40998=CIRCLE ( 'NONE', #45190, 0.09999999999999999167 ) ;
#40999=AXIS2_PLACEMENT_3D ( 'NONE', #90485, #97255, #829 ) ;
#41001=CARTESIAN_POINT ( 'NONE',  ( -12.69999999999999218, 12.50000000000000000, -0.4115034346978115321 ) ) ;
#41002=ORIENTED_EDGE ( 'NONE', *, *, #95906, .F. ) ;
#41003=EDGE_CURVE ( 'NONE', #101165, #85897, #100665, .T. ) ;
#41004=ORIENTED_EDGE ( 'NONE', *, *, #1060, .F. ) ;
#41005=EDGE_CURVE ( 'NONE', #26724, #54326, #119040, .T. ) ;
#41007=DIRECTION ( 'NONE',  ( 0.000000000000000000, 0.000000000000000000, -1.000000000000000000 ) ) ;
#41008=CARTESIAN_POINT ( 'NONE',  ( 1.849999999999950129, 2.500000000000000000, -6.841600689897078702 ) ) ;
#41009=DIRECTION ( 'NONE',  ( 0.000000000000000000, 1.000000000000000000, 0.000000000000000000 ) ) ;
#41010=EDGE_CURVE ( 'NONE', #70210, #61697, #110501, .T. ) ;
#41011=DIRECTION ( 'NONE',  ( 0.000000000000000000, 0.000000000000000000, 1.000000000000000000 ) ) ;
#41012=CARTESIAN_POINT ( 'NONE',  ( 11.24999999999994493, 2.500000000000000000, -2.065063509461102065 ) ) ;
#41013=CARTESIAN_POINT ( 'NONE',  ( 14.14999999999989377, 12.50000000000000000, -1.472243186433550122 ) ) ;
#41014=CIRCLE ( 'NONE', #72298, 0.06509327318403745899 ) ;
#41015=CARTESIAN_POINT ( 'NONE',  ( 13.94999999999989804, 2.500000000000000000, 1.818653347947321475 ) ) ;
#41016=DIRECTION ( 'NONE',  ( 0.000000000000000000, 1.000000000000000000, 0.000000000000000000 ) ) ;
#41017=CARTESIAN_POINT ( 'NONE',  ( -2.900000000000029221, 2.500000000000000000, -4.430127018922202176 ) ) ;
#41018=ORIENTED_EDGE ( 'NONE', *, *, #108766, .T. ) ;
#41019=CARTESIAN_POINT ( 'NONE',  ( 6.449999999999933564, 12.50000000000000000, -6.841600689897078702 ) ) ;
#41020=DIRECTION ( 'NONE',  ( 0.000000000000000000, 0.000000000000000000, 1.000000000000000000 ) ) ;
#41022=DIRECTION ( 'NONE',  ( 0.000000000000000000, 1.000000000000000000, 0.000000000000000000 ) ) ;
#41023=ORIENTED_EDGE ( 'NONE', *, *, #81030, .F. ) ;
#41024=CARTESIAN_POINT ( 'NONE',  ( 8.349999999999923261, 2.500000000000000000, 2.165063509461097713 ) ) ;
#41025=CONICAL_SURFACE ( 'NONE', #51478, 0.1000000000000002554, 0.003490658503988666988 ) ;
#41026=CIRCLE ( 'NONE', #30564, 0.06509327318403745899 ) ;
#41027=DIRECTION ( 'NONE',  ( 0.000000000000000000, 1.000000000000000000, 0.000000000000000000 ) ) ;
#41028=CARTESIAN_POINT ( 'NONE',  ( 11.24999999999990763, 2.500000000000000000, 1.572243186433545548 ) ) ;
#41029=ORIENTED_EDGE ( 'NONE', *, *, #480, .T. ) ;
#41031=EDGE_CURVE ( 'NONE', #23794, #17700, #19300, .T. ) ;
#41032=VERTEX_POINT ( 'NONE', #67990 ) ;
#41033=CIRCLE ( 'NONE', #34769, 0.06509327318403745899 ) ;
#41034=DIRECTION ( 'NONE',  ( 0.000000000000000000, 0.000000000000000000, 1.000000000000000000 ) ) ;
#41035=EDGE_LOOP ( 'NONE', ( #95054, #123961, #58791, #11333 ) ) ;
#41036=EDGE_LOOP ( 'NONE', ( #10362, #81350, #23148, #44027 ) ) ;
#41037=FACE_OUTER_BOUND ( 'NONE', #60945, .T. ) ;
#41038=EDGE_CURVE ( 'NONE', #123828, #83387, #54903, .T. ) ;
#41039=ADVANCED_FACE ( 'NONE', ( #29382 ), #89575, .T. ) ;
#41040=CARTESIAN_POINT ( 'NONE',  ( 5.849999999999933031, 2.500000000000000000, -1.372243186433550033 ) ) ;
#41041=CARTESIAN_POINT ( 'NONE',  ( -6.050000000000020250, 2.500000000000000000, -6.941600689897078347 ) ) ;
#41042=EDGE_CURVE ( 'NONE', #117955, #71169, #13029, .T. ) ;
#41043=CIRCLE ( 'NONE', #57757, 0.09999999999999982514 ) ;
#41044=AXIS2_PLACEMENT_3D ( 'NONE', #30912, #110734, #2064 ) ;
#41045=DIRECTION ( 'NONE',  ( 0.000000000000000000, 0.000000000000000000, -1.000000000000000000 ) ) ;
#41046=ORIENTED_EDGE ( 'NONE', *, *, #1179, .F. ) ;
#41047=CONICAL_SURFACE ( 'NONE', #18023, 0.1000000000000002554, 0.003490658503988666988 ) ;
#41048=DIRECTION ( 'NONE',  ( 0.000000000000000000, 0.000000000000000000, 1.000000000000000000 ) ) ;
#41049=ORIENTED_EDGE ( 'NONE', *, *, #41158, .F. ) ;
#41050=ADVANCED_FACE ( 'NONE', ( #19542 ), #46594, .T. ) ;
#41052=EDGE_CURVE ( 'NONE', #120493, #112688, #27805, .T. ) ;
#41053=CARTESIAN_POINT ( 'NONE',  ( 0.8499999999999536815, 2.500000000000000000, 5.802370205355744659 ) ) ;
#41054=ADVANCED_FACE ( 'NONE', ( #109868 ), #40359, .T. ) ;
#41055=ORIENTED_EDGE ( 'NONE', *, *, #75443, .T. ) ;
#41056=EDGE_CURVE ( 'NONE', #63798, #11368, #57049, .T. ) ;
#41057=EDGE_CURVE ( 'NONE', #24974, #68058, #50300, .T. ) ;
#41058=EDGE_LOOP ( 'NONE', ( #46176, #17582 ) ) ;
#41059=ORIENTED_EDGE ( 'NONE', *, *, #64408, .F. ) ;
#41060=EDGE_LOOP ( 'NONE', ( #38844, #75658 ) ) ;
#41061=DIRECTION ( 'NONE',  ( 0.000000000000000000, -0.000000000000000000, 1.000000000000000000 ) ) ;
#41062=CARTESIAN_POINT ( 'NONE',  ( 9.112263991835201082, 1.500000000000000222, 9.392448311626331758 ) ) ;
#41063=CARTESIAN_POINT ( 'NONE',  ( 4.599999999999936584, 2.500000000000000000, 4.330127018922196314 ) ) ;
#41064=FACE_BOUND ( 'NONE', #122014, .T. ) ;
#41065=CARTESIAN_POINT ( 'NONE',  ( -2.900000000000030109, 2.500000000000000000, -3.637306695894650055 ) ) ;
#41066=AXIS2_PLACEMENT_3D ( 'NONE', #29348, #39818, #69239 ) ;
#41068=EDGE_CURVE ( 'NONE', #57799, #19758, #73778, .T. ) ;
#41069=CARTESIAN_POINT ( 'NONE',  ( 6.849999999999930367, 2.500000000000000000, -6.248780366869526759 ) ) ;
#41070=DIRECTION ( 'NONE',  ( 0.000000000000000000, 0.000000000000000000, -1.000000000000000000 ) ) ;
#41071=PLANE ( 'NONE',  #90337 ) ;
#41072=AXIS2_PLACEMENT_3D ( 'NONE', #17566, #67959, #56203 ) ;
#41073=DIRECTION ( 'NONE',  ( 0.000000000000000000, 1.000000000000000000, 0.000000000000000000 ) ) ;
#41074=DIRECTION ( 'NONE',  ( -0.000000000000000000, 1.000000000000000000, -0.000000000000000000 ) ) ;
#41075=AXIS2_PLACEMENT_3D ( 'NONE', #100614, #81626, #12235 ) ;
#41076=VECTOR ( 'NONE', #119290, 1000.000000000000000 ) ;
#41077=CARTESIAN_POINT ( 'NONE',  ( 11.89999999999990798, 2.500000000000000000, -4.576537180435977348 ) ) ;
#41078=AXIS2_PLACEMENT_3D ( 'NONE', #45735, #126872, #35906 ) ;
#41079=ORIENTED_EDGE ( 'NONE', *, *, #119425, .F. ) ;
#41080=ORIENTED_EDGE ( 'NONE', *, *, #89569, .T. ) ;
#41081=VERTEX_POINT ( 'NONE', #60141 ) ;
#41082=EDGE_LOOP ( 'NONE', ( #57184, #125171 ) ) ;
#41083=VERTEX_POINT ( 'NONE', #28081 ) ;
#41085=DIRECTION ( 'NONE',  ( 0.000000000000000000, 1.000000000000000000, 0.000000000000000000 ) ) ;
#41086=ORIENTED_EDGE ( 'NONE', *, *, #30656, .F. ) ;
#41087=FACE_BOUND ( 'NONE', #116870, .T. ) ;
#41088=AXIS2_PLACEMENT_3D ( 'NONE', #24458, #111040, #45397 ) ;
#41089=PLANE ( 'NONE',  #66638 ) ;
#41091=VECTOR ( 'NONE', #44626, 1000.000000000000000 ) ;
#41092=ORIENTED_EDGE ( 'NONE', *, *, #105541, .T. ) ;
#41093=LINE ( 'NONE', #71165, #65674 ) ;
#41094=DIRECTION ( 'NONE',  ( 0.000000000000000000, 0.000000000000000000, 1.000000000000000000 ) ) ;
#41095=CARTESIAN_POINT ( 'NONE',  ( -13.74999999999995381, 2.500000000000000000, -2.065063509461099844 ) ) ;
#41096=DIRECTION ( 'NONE',  ( -0.000000000000000000, 1.000000000000000000, -0.000000000000000000 ) ) ;
#41097=EDGE_LOOP ( 'NONE', ( #55106, #110945 ) ) ;
#41098=DIRECTION ( 'NONE',  ( 0.000000000000000000, 1.000000000000000000, 0.000000000000000000 ) ) ;
#41099=ADVANCED_FACE ( 'NONE', ( #18250 ), #117668, .T. ) ;
#41100=ORIENTED_EDGE ( 'NONE', *, *, #1476, .F. ) ;
#41101=ORIENTED_EDGE ( 'NONE', *, *, #66676, .T. ) ;
#41102=CARTESIAN_POINT ( 'NONE',  ( 1.249999999999954259, 2.500000000000000000, -7.288010851410854585 ) ) ;
#41103=CARTESIAN_POINT ( 'NONE',  ( 3.949999999999942446, 12.50000000000000000, -6.906693963081115939 ) ) ;
#41104=ORIENTED_EDGE ( 'NONE', *, *, #61378, .T. ) ;
#41105=CARTESIAN_POINT ( 'NONE',  ( 11.64999999999990621, 12.50000000000000000, 6.560283801567334372 ) ) ;
#41106=DIRECTION ( 'NONE',  ( -0.000000000000000000, -1.000000000000000000, -0.000000000000000000 ) ) ;
#41107=PLANE ( 'NONE',  #33183 ) ;
#41108=DIRECTION ( 'NONE',  ( 0.000000000000000000, 0.000000000000000000, 1.000000000000000000 ) ) ;
#41109=EDGE_LOOP ( 'NONE', ( #68134, #11217, #100187, #815 ) ) ;
#41110=ADVANCED_FACE ( 'NONE', ( #48360 ), #42407, .T. ) ;
#41111=DIRECTION ( 'NONE',  ( 0.000000000000000000, -0.000000000000000000, 1.000000000000000000 ) ) ;
#41112=ORIENTED_EDGE ( 'NONE', *, *, #99912, .T. ) ;
#41113=CARTESIAN_POINT ( 'NONE',  ( 11.24999999999994316, 2.500000000000000000, 2.165063509461097713 ) ) ;
#41114=CIRCLE ( 'NONE', #28578, 0.1000000000000002554 ) ;
#41115=EDGE_LOOP ( 'NONE', ( #36470, #31808, #107502, #22533 ) ) ;
#41116=VECTOR ( 'NONE', #103463, 1000.000000000000000 ) ;
#41117=CARTESIAN_POINT ( 'NONE',  ( -1.050000000000037792, 2.500000000000000000, 1.818653347947321475 ) ) ;
#41118=EDGE_LOOP ( 'NONE', ( #125773, #117496, #24012, #116080 ) ) ;
#41119=FACE_OUTER_BOUND ( 'NONE', #20242, .T. ) ;
#41120=DIRECTION ( 'NONE',  ( 0.000000000000000000, 0.000000000000000000, 1.000000000000000000 ) ) ;
#41121=DIRECTION ( 'NONE',  ( 0.000000000000000000, 1.000000000000000000, 0.000000000000000000 ) ) ;
#41122=CARTESIAN_POINT ( 'NONE',  ( 13.09999999999990195, 2.500000000000000000, -4.576537180435978236 ) ) ;
#41123=CARTESIAN_POINT ( 'NONE',  ( -9.400000000000009237, 2.500000000000000000, -4.576537180435973795 ) ) ;
#41124=EDGE_LOOP ( 'NONE', ( #75075, #112180 ) ) ;
#41125=AXIS2_PLACEMENT_3D ( 'NONE', #91073, #70157, #41354 ) ;
#41126=VERTEX_POINT ( 'NONE', #119670 ) ;
#41127=ORIENTED_EDGE ( 'NONE', *, *, #113243, .F. ) ;
#41128=DIRECTION ( 'NONE',  ( 0.000000000000000000, 0.000000000000000000, 1.000000000000000000 ) ) ;
#41129=DIRECTION ( 'NONE',  ( 0.000000000000000000, 1.000000000000000000, 0.000000000000000000 ) ) ;
#41130=CARTESIAN_POINT ( 'NONE',  ( -11.24999999999996270, 2.500000000000000000, 2.065063509461097624 ) ) ;
#41131=VERTEX_POINT ( 'NONE', #8421 ) ;
#41132=ORIENTED_EDGE ( 'NONE', *, *, #105328, .F. ) ;
#41133=ORIENTED_EDGE ( 'NONE', *, *, #61964, .T. ) ;
#41134=DIRECTION ( 'NONE',  ( 0.000000000000000000, 0.000000000000000000, 1.000000000000000000 ) ) ;
#41135=AXIS2_PLACEMENT_3D ( 'NONE', #83807, #84463, #3323 ) ;
#41136=VERTEX_POINT ( 'NONE', #88261 ) ;
#41137=FACE_OUTER_BOUND ( 'NONE', #114269, .T. ) ;
#41138=DIRECTION ( 'NONE',  ( -0.000000000000000000, -1.000000000000000000, -0.000000000000000000 ) ) ;
#41139=VECTOR ( 'NONE', #37263, 1000.000000000000000 ) ;
#41140=EDGE_CURVE ( 'NONE', #6762, #39561, #30026, .T. ) ;
#41141=CARTESIAN_POINT ( 'NONE',  ( 3.299999999999944755, 2.500000000000000000, -4.230127018922201998 ) ) ;
#41142=CYLINDRICAL_SURFACE ( 'NONE', #8441, 7.500000000000000000 ) ;
#41143=DIRECTION ( 'NONE',  ( 0.000000000000000000, 0.000000000000000000, 1.000000000000000000 ) ) ;
#41144=DIRECTION ( 'NONE',  ( 0.000000000000000000, 0.000000000000000000, 1.000000000000000000 ) ) ;
#41145=CARTESIAN_POINT ( 'NONE',  ( 7.049999999999928768, 2.500000000000000000, -2.165063509461101710 ) ) ;
#41146=CARTESIAN_POINT ( 'NONE',  ( 13.34999999999989662, 12.50000000000000000, -2.165063509461101710 ) ) ;
#41147=EDGE_CURVE ( 'NONE', #14617, #125159, #63320, .T. ) ;
#41148=ORIENTED_EDGE ( 'NONE', *, *, #60509, .T. ) ;
#41149=DIRECTION ( 'NONE',  ( -4.274815082592931898E-19, -0.9999939076577903929, -0.003490651415223739937 ) ) ;
#41150=CARTESIAN_POINT ( 'NONE',  ( 10.19999999999991047, 2.500000000000000000, 4.776537180435972196 ) ) ;
#41151=EDGE_CURVE ( 'NONE', #34347, #64996, #21479, .T. ) ;
#41152=VERTEX_POINT ( 'NONE', #2462 ) ;
#41153=ADVANCED_FACE ( 'NONE', ( #120966 ), #113488, .T. ) ;
#41154=VERTEX_POINT ( 'NONE', #121599 ) ;
#41155=EDGE_CURVE ( 'NONE', #60040, #42741, #17321, .T. ) ;
#41157=CARTESIAN_POINT ( 'NONE',  ( 8.549999999999922551, 2.500000000000000000, 2.611473670974873151 ) ) ;
#41158=EDGE_CURVE ( 'NONE', #59648, #62565, #616, .T. ) ;
#41159=AXIS2_PLACEMENT_3D ( 'NONE', #76989, #34510, #54128 ) ;
#41160=EDGE_CURVE ( 'NONE', #26349, #38979, #34086, .T. ) ;
#41161=CARTESIAN_POINT ( 'NONE',  ( 11.64999999999990621, 2.500000000000000000, -2.165063509461101710 ) ) ;
#41163=AXIS2_PLACEMENT_3D ( 'NONE', #110151, #47366, #108207 ) ;
#41164=CARTESIAN_POINT ( 'NONE',  ( -9.800000000000006040, 2.500000000000000000, 4.676537180435972552 ) ) ;
#41165=CARTESIAN_POINT ( 'NONE',  ( -0.4500000000000402012, 2.500000000000000000, 6.495190528383297135 ) ) ;
#41166=CIRCLE ( 'NONE', #93370, 0.1000000000000002554 ) ;
#41167=CARTESIAN_POINT ( 'NONE',  ( -3.750000000000025757, 2.500000000000000000, -2.857883832488653741 ) ) ;
#41168=CARTESIAN_POINT ( 'NONE',  ( -6.850000000000013856, 12.50000000000000000, 6.841600689897072485 ) ) ;
#41169=EDGE_CURVE ( 'NONE', #118431, #90873, #15265, .T. ) ;
#41170=CIRCLE ( 'NONE', #85047, 0.1000000000000002554 ) ;
#41171=DIRECTION ( 'NONE',  ( 0.000000000000000000, -0.9999939076577903929, 0.003490651415223739937 ) ) ;
#41172=EDGE_CURVE ( 'NONE', #54506, #106259, #71883, .T. ) ;
#41173=ORIENTED_EDGE ( 'NONE', *, *, #89620, .F. ) ;
#41174=EDGE_CURVE ( 'NONE', #67575, #113131, #42423, .T. ) ;
#41175=ORIENTED_EDGE ( 'NONE', *, *, #74509, .T. ) ;
#41176=CIRCLE ( 'NONE', #76746, 0.1000000000000002554 ) ;
#41177=ORIENTED_EDGE ( 'NONE', *, *, #77983, .T. ) ;
#41178=EDGE_LOOP ( 'NONE', ( #80358, #110549 ) ) ;
#41179=CIRCLE ( 'NONE', #62095, 0.06509327318403745899 ) ;
#41180=EDGE_LOOP ( 'NONE', ( #14933, #55977 ) ) ;
#41181=DIRECTION ( 'NONE',  ( -4.274815082592931898E-19, -0.9999939076577903929, -0.003490651415223739937 ) ) ;
#41182=DIRECTION ( 'NONE',  ( -0.000000000000000000, -1.000000000000000000, -0.000000000000000000 ) ) ;
#41183=VECTOR ( 'NONE', #4148, 1000.000000000000000 ) ;
#41184=VERTEX_POINT ( 'NONE', #53527 ) ;
#41185=CARTESIAN_POINT ( 'NONE',  ( -15.59999999999998010, 2.500000000000000000, -0.2464101615137759549 ) ) ;
#41186=DIRECTION ( 'NONE',  ( -0.000000000000000000, 1.000000000000000000, -0.000000000000000000 ) ) ;
#41187=AXIS2_PLACEMENT_3D ( 'NONE', #21301, #111628, #61243 ) ;
#41188=CARTESIAN_POINT ( 'NONE',  ( 0.6499999999999543920, 12.50000000000000000, 6.841600689897072485 ) ) ;
#41189=FACE_OUTER_BOUND ( 'NONE', #3267, .T. ) ;
#41190=EDGE_LOOP ( 'NONE', ( #15277, #100072, #11418, #110214 ) ) ;
#41191=LINE ( 'NONE', #119713, #36904 ) ;
#41192=CARTESIAN_POINT ( 'NONE',  ( -8.150000000000012790, 2.500000000000000000, -2.511473670974877948 ) ) ;
#41193=VERTEX_POINT ( 'NONE', #10995 ) ;
#41194=ORIENTED_EDGE ( 'NONE', *, *, #49863, .T. ) ;
#41195=ORIENTED_EDGE ( 'NONE', *, *, #22832, .F. ) ;
#41196=ORIENTED_EDGE ( 'NONE', *, *, #12869, .T. ) ;
#41197=DIRECTION ( 'NONE',  ( 0.000000000000000000, 0.000000000000000000, 1.000000000000000000 ) ) ;
#41198=AXIS2_PLACEMENT_3D ( 'NONE', #76358, #116261, #26606 ) ;
#41199=DIRECTION ( 'NONE',  ( -0.000000000000000000, 1.000000000000000000, -0.000000000000000000 ) ) ;
#41200=DIRECTION ( 'NONE',  ( -0.000000000000000000, 1.000000000000000000, -0.000000000000000000 ) ) ;
#41201=FACE_OUTER_BOUND ( 'NONE', #28795, .T. ) ;
#41202=EDGE_LOOP ( 'NONE', ( #31483, #120074 ) ) ;
#41203=FACE_OUTER_BOUND ( 'NONE', #45752, .T. ) ;
#41204=CARTESIAN_POINT ( 'NONE',  ( -7.050000000000013145, 2.500000000000000000, 6.395190528383296602 ) ) ;
#41205=DIRECTION ( 'NONE',  ( 0.000000000000000000, 1.000000000000000000, 0.000000000000000000 ) ) ;
#41206=DIRECTION ( 'NONE',  ( 0.000000000000000000, 1.000000000000000000, 0.000000000000000000 ) ) ;
#41207=ADVANCED_FACE ( 'NONE', ( #90862 ), #48758, .T. ) ;
#41208=EDGE_CURVE ( 'NONE', #109623, #100170, #82352, .T. ) ;
#41209=ORIENTED_EDGE ( 'NONE', *, *, #92992, .F. ) ;
#41210=VECTOR ( 'NONE', #96779, 1000.000000000000000 ) ;
#41211=AXIS2_PLACEMENT_3D ( 'NONE', #30409, #67715, #129258 ) ;
#41212=EDGE_CURVE ( 'NONE', #54324, #66570, #107230, .T. ) ;
#41213=EDGE_LOOP ( 'NONE', ( #54822, #119634 ) ) ;
#41214=ORIENTED_EDGE ( 'NONE', *, *, #92085, .T. ) ;
#41215=DIRECTION ( 'NONE',  ( 0.000000000000000000, 0.000000000000000000, 1.000000000000000000 ) ) ;
#41216=DIRECTION ( 'NONE',  ( -0.000000000000000000, 1.000000000000000000, -0.000000000000000000 ) ) ;
#41217=FACE_BOUND ( 'NONE', #124115, .T. ) ;
#41218=CARTESIAN_POINT ( 'NONE',  ( 13.34999999999989662, 2.500000000000000000, -2.265063509461101798 ) ) ;
#41219=DIRECTION ( 'NONE',  ( -0.000000000000000000, 1.000000000000000000, -0.000000000000000000 ) ) ;
#41220=EDGE_CURVE ( 'NONE', #71397, #88786, #50813, .T. ) ;
#41221=VECTOR ( 'NONE', #49087, 1000.000000000000000 ) ;
#41222=CIRCLE ( 'NONE', #16126, 0.1000000000000002554 ) ;
#41223=CARTESIAN_POINT ( 'NONE',  ( -4.350000000000027178, 2.500000000000000000, -6.248780366869526759 ) ) ;
#41224=CARTESIAN_POINT ( 'NONE',  ( -12.09999999999999609, 2.500000000000000000, -5.122947341949751987 ) ) ;
#41225=FACE_OUTER_BOUND ( 'NONE', #19175, .T. ) ;
#41226=DIRECTION ( 'NONE',  ( 0.000000000000000000, 0.000000000000000000, 1.000000000000000000 ) ) ;
#41227=EDGE_LOOP ( 'NONE', ( #56560, #110413 ) ) ;
#41228=AXIS2_PLACEMENT_3D ( 'NONE', #99925, #102496, #69816 ) ;
#41229=DIRECTION ( 'NONE',  ( 0.000000000000000000, 0.000000000000000000, 1.000000000000000000 ) ) ;
#41230=CARTESIAN_POINT ( 'NONE',  ( 9.999999999999912959, 2.500000000000000000, 3.637306695894644726 ) ) ;
#41231=ORIENTED_EDGE ( 'NONE', *, *, #113389, .T. ) ;
#41232=VERTEX_POINT ( 'NONE', #43084 ) ;
#41233=FACE_OUTER_BOUND ( 'NONE', #59110, .T. ) ;
#41234=CARTESIAN_POINT ( 'NONE',  ( 9.149999999999920419, 12.50000000000000000, -7.122917578226816815 ) ) ;
#41236=FACE_BOUND ( 'NONE', #27574, .T. ) ;
#41237=CARTESIAN_POINT ( 'NONE',  ( 2.099999999999948574, 12.50000000000000000, 4.265033745738159077 ) ) ;
#41238=FACE_OUTER_BOUND ( 'NONE', #49521, .T. ) ;
#41239=VERTEX_POINT ( 'NONE', #22791 ) ;
#41240=DIRECTION ( 'NONE',  ( -0.000000000000000000, -1.000000000000000000, -0.000000000000000000 ) ) ;
#41242=AXIS2_PLACEMENT_3D ( 'NONE', #29502, #10487, #70708 ) ;
#41243=ORIENTED_EDGE ( 'NONE', *, *, #63912, .F. ) ;
#41244=DIRECTION ( 'NONE',  ( 0.000000000000000000, 0.000000000000000000, 1.000000000000000000 ) ) ;
#41245=CONICAL_SURFACE ( 'NONE', #101867, 0.1000000000000002554, 0.003490658503988666988 ) ;
#41246=DIRECTION ( 'NONE',  ( -1.000000000000000000, -0.000000000000000000, -0.000000000000000000 ) ) ;
#41247=AXIS2_PLACEMENT_3D ( 'NONE', #84003, #93840, #84662 ) ;
#41248=EDGE_CURVE ( 'NONE', #57762, #114896, #92565, .T. ) ;
#41249=CARTESIAN_POINT ( 'NONE',  ( -2.100000000000033840, 2.500000000000000000, 3.637306695894644726 ) ) ;
#41250=LINE ( 'NONE', #121716, #86573 ) ;
#41251=VECTOR ( 'NONE', #95812, 1000.000000000000000 ) ;
#41252=ORIENTED_EDGE ( 'NONE', *, *, #2983, .F. ) ;
#41253=AXIS2_PLACEMENT_3D ( 'NONE', #36684, #107335, #66118 ) ;
#41254=CARTESIAN_POINT ( 'NONE',  ( 11.24999999999990585, 2.500000000000000000, -5.702370205355749455 ) ) ;
#41255=CARTESIAN_POINT ( 'NONE',  ( -12.49999999999999467, 2.500000000000000000, 0.6928203230275535862 ) ) ;
#41256=CARTESIAN_POINT ( 'NONE',  ( 4.399999999999937295, 2.500000000000000000, 4.776537180435972196 ) ) ;
#41257=ORIENTED_EDGE ( 'NONE', *, *, #38427, .T. ) ;
#41258=ORIENTED_EDGE ( 'NONE', *, *, #32348, .T. ) ;
#41259=CIRCLE ( 'NONE', #85146, 0.06509327318403745899 ) ;
#41260=ADVANCED_FACE ( 'NONE', ( #113072 ), #32045, .T. ) ;
#41262=LINE ( 'NONE', #51716, #7495 ) ;
#41263=ORIENTED_EDGE ( 'NONE', *, *, #38307, .F. ) ;
#41264=DIRECTION ( 'NONE',  ( 0.000000000000000000, 0.000000000000000000, 1.000000000000000000 ) ) ;
#41265=DIRECTION ( 'NONE',  ( 0.000000000000000000, 0.000000000000000000, 1.000000000000000000 ) ) ;
#41266=AXIS2_PLACEMENT_3D ( 'NONE', #108877, #67668, #97142 ) ;
#41267=CIRCLE ( 'NONE', #124878, 0.1000000000000002554 ) ;
#41268=DIRECTION ( 'NONE',  ( -4.274815082592931898E-19, -0.9999939076577903929, -0.003490651415223739937 ) ) ;
#41269=ORIENTED_EDGE ( 'NONE', *, *, #112257, .F. ) ;
#41270=PLANE ( 'NONE',  #5703 ) ;
#41271=FACE_OUTER_BOUND ( 'NONE', #14682, .T. ) ;
#41272=LINE ( 'NONE', #117863, #105013 ) ;
#41273=CARTESIAN_POINT ( 'NONE',  ( -1.050000000000038236, 2.500000000000000000, -1.918653347947326004 ) ) ;
#41274=DIRECTION ( 'NONE',  ( 0.000000000000000000, 1.000000000000000000, 0.000000000000000000 ) ) ;
#41275=CARTESIAN_POINT ( 'NONE',  ( -11.89999999999999680, 12.50000000000000000, -4.676537180435976104 ) ) ;
#41276=EDGE_LOOP ( 'NONE', ( #40181, #120314, #28938, #1123 ) ) ;
#41277=ORIENTED_EDGE ( 'NONE', *, *, #66099, .F. ) ;
#41278=DIRECTION ( 'NONE',  ( 0.000000000000000000, 1.000000000000000000, 0.000000000000000000 ) ) ;
#41279=ORIENTED_EDGE ( 'NONE', *, *, #107933, .F. ) ;
#41280=DIRECTION ( 'NONE',  ( -4.274815082592931898E-19, -0.9999939076577903929, -0.003490651415223739937 ) ) ;
#41281=EDGE_LOOP ( 'NONE', ( #19832, #14094, #70699, #47544 ) ) ;
#41282=ORIENTED_EDGE ( 'NONE', *, *, #1550, .F. ) ;
#41283=ORIENTED_EDGE ( 'NONE', *, *, #56687, .T. ) ;
#41284=AXIS2_PLACEMENT_3D ( 'NONE', #16882, #14326, #15618 ) ;
#41285=LINE ( 'NONE', #53661, #85556 ) ;
#41286=DIRECTION ( 'NONE',  ( -0.000000000000000000, -1.000000000000000000, -0.000000000000000000 ) ) ;
#41287=DIRECTION ( 'NONE',  ( -0.000000000000000000, -1.000000000000000000, -0.000000000000000000 ) ) ;
#41288=EDGE_CURVE ( 'NONE', #3112, #111831, #61279, .T. ) ;
#41289=DIRECTION ( 'NONE',  ( 0.000000000000000000, -0.9999939076577903929, 0.003490651415223739937 ) ) ;
#41290=CARTESIAN_POINT ( 'NONE',  ( -5.400000000000019895, 12.50000000000000000, -0.6928203230275541413 ) ) ;
#41292=FACE_OUTER_BOUND ( 'NONE', #78652, .T. ) ;
#41293=CARTESIAN_POINT ( 'NONE',  ( 5.449999999999937117, 2.500000000000000000, -6.495190528383302464 ) ) ;
#41294=DIRECTION ( 'NONE',  ( 0.000000000000000000, 1.000000000000000000, 0.000000000000000000 ) ) ;
#41295=EDGE_CURVE ( 'NONE', #85147, #31487, #126000, .T. ) ;
#41297=VERTEX_POINT ( 'NONE', #18671 ) ;
#41298=CIRCLE ( 'NONE', #126965, 0.06509327318403745899 ) ;
#41299=CARTESIAN_POINT ( 'NONE',  ( -0.6500000000000394351, 12.50000000000000000, 2.511473670974873507 ) ) ;
#41300=ADVANCED_FACE ( 'NONE', ( #58611 ), #99824, .T. ) ;
#41301=VERTEX_POINT ( 'NONE', #38996 ) ;
#41302=EDGE_CURVE ( 'NONE', #66032, #112123, #96752, .T. ) ;
#41303=ORIENTED_EDGE ( 'NONE', *, *, #23535, .F. ) ;
#41304=EDGE_CURVE ( 'NONE', #22551, #82878, #77992, .T. ) ;
#41305=DIRECTION ( 'NONE',  ( 0.000000000000000000, 0.000000000000000000, -1.000000000000000000 ) ) ;
#41306=ADVANCED_FACE ( 'NONE', ( #119436 ), #59915, .T. ) ;
#41307=FACE_OUTER_BOUND ( 'NONE', #118539, .T. ) ;
#41308=CIRCLE ( 'NONE', #76796, 0.06509327318403745899 ) ;
#41309=VECTOR ( 'NONE', #126811, 1000.000000000000000 ) ;
#41310=CARTESIAN_POINT ( 'NONE',  ( -12.89999999999999147, 2.500000000000000000, -5.022947341949751454 ) ) ;
#41311=CARTESIAN_POINT ( 'NONE',  ( 1.649999999999949729, 12.50000000000000000, 5.802370205355744659 ) ) ;
#41312=DIRECTION ( 'NONE',  ( 0.000000000000000000, 1.000000000000000000, 0.000000000000000000 ) ) ;
#41313=EDGE_CURVE ( 'NONE', #74338, #31381, #109287, .T. ) ;
#41314=CARTESIAN_POINT ( 'NONE',  ( -11.44999999999999751, 2.500000000000000000, -2.511473670974873951 ) ) ;
#41315=ORIENTED_EDGE ( 'NONE', *, *, #101275, .T. ) ;
#41316=ADVANCED_FACE ( 'NONE', ( #69709 ), #119849, .T. ) ;
#41317=EDGE_CURVE ( 'NONE', #114882, #80384, #29879, .T. ) ;
#41318=AXIS2_PLACEMENT_3D ( 'NONE', #117432, #106357, #38273 ) ;
#41319=EDGE_CURVE ( 'NONE', #92599, #45421, #107326, .T. ) ;
#41320=ORIENTED_EDGE ( 'NONE', *, *, #63860, .T. ) ;
#41321=VECTOR ( 'NONE', #120595, 1000.000000000000000 ) ;
#41322=EDGE_CURVE ( 'NONE', #59852, #109430, #78257, .T. ) ;
#41323=ORIENTED_EDGE ( 'NONE', *, *, #2352, .F. ) ;
#41324=DIRECTION ( 'NONE',  ( 0.000000000000000000, 1.000000000000000000, 0.000000000000000000 ) ) ;
#41325=VERTEX_POINT ( 'NONE', #50095 ) ;
#41326=ORIENTED_EDGE ( 'NONE', *, *, #32501, .F. ) ;
#41327=EDGE_CURVE ( 'NONE', #107807, #17323, #71004, .T. ) ;
#41328=DIRECTION ( 'NONE',  ( -4.274815082592931898E-19, -0.9999939076577903929, -0.003490651415223739937 ) ) ;
#41329=DIRECTION ( 'NONE',  ( 0.000000000000000000, 0.000000000000000000, 1.000000000000000000 ) ) ;
#41330=AXIS2_PLACEMENT_3D ( 'NONE', #74893, #6753, #96441 ) ;
#41331=DIRECTION ( 'NONE',  ( -0.000000000000000000, -1.000000000000000000, -0.000000000000000000 ) ) ;
#41332=LINE ( 'NONE', #51780, #79973 ) ;
#41333=CARTESIAN_POINT ( 'NONE',  ( 17.50000000000000000, -2.500000000000000000, 4.000000000000001776 ) ) ;
#41334=ORIENTED_EDGE ( 'NONE', *, *, #75222, .F. ) ;
#41335=CARTESIAN_POINT ( 'NONE',  ( 6.849999999999929479, 2.500000000000000000, -2.511473670974877948 ) ) ;
#41336=DIRECTION ( 'NONE',  ( 0.000000000000000000, 0.000000000000000000, -1.000000000000000000 ) ) ;
#41337=CARTESIAN_POINT ( 'NONE',  ( -4.550000000000026468, 12.50000000000000000, -6.495190528383302464 ) ) ;
#41338=CARTESIAN_POINT ( 'NONE',  ( 4.149999999999941735, 2.500000000000000000, -5.802370205355749988 ) ) ;
#41339=AXIS2_PLACEMENT_3D ( 'NONE', #58806, #40469, #79102 ) ;
#41340=AXIS2_PLACEMENT_3D ( 'NONE', #97369, #108471, #18799 ) ;
#41341=DIRECTION ( 'NONE',  ( 0.000000000000000000, 0.000000000000000000, -1.000000000000000000 ) ) ;
#41342=ORIENTED_EDGE ( 'NONE', *, *, #46752, .T. ) ;
#41343=CIRCLE ( 'NONE', #45446, 0.06509327318403745899 ) ;
#41344=VERTEX_POINT ( 'NONE', #40258 ) ;
#41345=ORIENTED_EDGE ( 'NONE', *, *, #20910, .F. ) ;
#41347=AXIS2_PLACEMENT_3D ( 'NONE', #43997, #111416, #13217 ) ;
#41348=VERTEX_POINT ( 'NONE', #98502 ) ;
#41349=AXIS2_PLACEMENT_3D ( 'NONE', #22594, #33055, #992 ) ;
#41350=CARTESIAN_POINT ( 'NONE',  ( 16.89731025888664462, -0.9183091266721399304, 5.698390440797583167 ) ) ;
#41351=LINE ( 'NONE', #91716, #29332 ) ;
#41352=AXIS2_PLACEMENT_3D ( 'NONE', #120391, #21541, #10426 ) ;
#41353=VERTEX_POINT ( 'NONE', #8837 ) ;
#41354=DIRECTION ( 'NONE',  ( 0.000000000000000000, 0.000000000000000000, -1.000000000000000000 ) ) ;
#41355=CARTESIAN_POINT ( 'NONE',  ( 6.249999999999928946, 12.50000000000000000, 2.857883832488649301 ) ) ;
#41356=CIRCLE ( 'NONE', #114484, 0.06509327318403745899 ) ;
#41357=DIRECTION ( 'NONE',  ( -0.000000000000000000, 1.000000000000000000, -0.000000000000000000 ) ) ;
#41358=DIRECTION ( 'NONE',  ( 0.000000000000000000, 1.000000000000000000, 0.000000000000000000 ) ) ;
#41359=ADVANCED_FACE ( 'NONE', ( #48792 ), #80177, .T. ) ;
#41361=AXIS2_PLACEMENT_3D ( 'NONE', #119904, #99627, #40724 ) ;
#41362=FACE_OUTER_BOUND ( 'NONE', #84385, .T. ) ;
#41363=EDGE_CURVE ( 'NONE', #30275, #29752, #122003, .T. ) ;
#41364=ORIENTED_EDGE ( 'NONE', *, *, #58774, .T. ) ;
#41365=ORIENTED_EDGE ( 'NONE', *, *, #31586, .F. ) ;
#41366=DIRECTION ( 'NONE',  ( 0.000000000000000000, 1.000000000000000000, 0.000000000000000000 ) ) ;
#41367=CARTESIAN_POINT ( 'NONE',  ( 3.549999999999942979, 2.500000000000000000, 1.818653347947321475 ) ) ;
#41368=CARTESIAN_POINT ( 'NONE',  ( 1.449999999999951328, 2.500000000000000000, 2.411473670974873862 ) ) ;
#41369=ADVANCED_FACE ( 'NONE', ( #50711 ), #84344, .T. ) ;
#41370=DIRECTION ( 'NONE',  ( 0.000000000000000000, -0.000000000000000000, 1.000000000000000000 ) ) ;
#41371=ORIENTED_EDGE ( 'NONE', *, *, #5384, .F. ) ;
#41372=VERTEX_POINT ( 'NONE', #110905 ) ;
#41373=DIRECTION ( 'NONE',  ( 0.000000000000000000, 0.000000000000000000, -1.000000000000000000 ) ) ;
#41374=CARTESIAN_POINT ( 'NONE',  ( -13.09999999999999254, 12.50000000000000000, -4.611443907251937091 ) ) ;
#41375=CARTESIAN_POINT ( 'NONE',  ( 0.5999999999999547917, 2.500000000000000000, 3.983716857408420076 ) ) ;
#41377=ORIENTED_EDGE ( 'NONE', *, *, #9682, .F. ) ;
#41378=CARTESIAN_POINT ( 'NONE',  ( 0.4499999999999573785, 12.50000000000000000, -6.495190528383302464 ) ) ;
#41379=DIRECTION ( 'NONE',  ( -0.000000000000000000, -1.000000000000000000, -0.000000000000000000 ) ) ;
#41380=EDGE_LOOP ( 'NONE', ( #112868, #25580, #3949, #30135 ) ) ;
#41381=CARTESIAN_POINT ( 'NONE',  ( 17.50000000000000000, 2.500000000000000000, 2.922290670087886344 ) ) ;
#41382=ORIENTED_EDGE ( 'NONE', *, *, #101984, .F. ) ;
#41383=DIRECTION ( 'NONE',  ( -4.274815082592931898E-19, -0.9999939076577903929, -0.003490651415223739937 ) ) ;
#41384=AXIS2_PLACEMENT_3D ( 'NONE', #63005, #90523, #102921 ) ;
#41385=ORIENTED_EDGE ( 'NONE', *, *, #127999, .T. ) ;
#41386=AXIS2_PLACEMENT_3D ( 'NONE', #30253, #47944, #108775 ) ;
#41387=ORIENTED_EDGE ( 'NONE', *, *, #4228, .T. ) ;
#41388=LINE ( 'NONE', #79373, #113302 ) ;
#41389=DIRECTION ( 'NONE',  ( -0.000000000000000000, 1.000000000000000000, -0.000000000000000000 ) ) ;
#41390=ORIENTED_EDGE ( 'NONE', *, *, #4668, .F. ) ;
#41391=EDGE_LOOP ( 'NONE', ( #79356, #25237 ) ) ;
#41392=CARTESIAN_POINT ( 'NONE',  ( -9.550000000000007816, 12.50000000000000000, -6.495190528383297135 ) ) ;
#41393=CARTESIAN_POINT ( 'NONE',  ( -1.850000000000033396, 12.50000000000000000, -1.883746621131363375 ) ) ;
#41394=ORIENTED_EDGE ( 'NONE', *, *, #101029, .F. ) ;
#41395=AXIS2_PLACEMENT_3D ( 'NONE', #122434, #22316, #83159 ) ;
#41396=DIRECTION ( 'NONE',  ( 0.000000000000000000, -0.9999939076577903929, 0.003490651415223739937 ) ) ;
#41397=ADVANCED_FACE ( 'NONE', ( #21243 ), #61181, .T. ) ;
#41399=CIRCLE ( 'NONE', #51854, 0.06509327318403745899 ) ;
#41400=CARTESIAN_POINT ( 'NONE',  ( -5.400000000000023448, 2.500000000000000000, -4.230127018922201998 ) ) ;
#41401=CARTESIAN_POINT ( 'NONE',  ( 13.14999999999990088, 2.500000000000000000, 1.718653347947321386 ) ) ;
#41402=CARTESIAN_POINT ( 'NONE',  ( -9.600000000000008527, 2.500000000000000000, -4.330127018922197202 ) ) ;
#41403=CARTESIAN_POINT ( 'NONE',  ( 14.14999999999989733, 2.500000000000000000, 2.857883832488649301 ) ) ;
#41404=DIRECTION ( 'NONE',  ( -4.274815082592931898E-19, -0.9999939076577903929, -0.003490651415223739937 ) ) ;
#41405=CONICAL_SURFACE ( 'NONE', #51860, 0.1000000000000002554, 0.003490658503988666988 ) ;
#41406=ORIENTED_EDGE ( 'NONE', *, *, #37621, .F. ) ;
#41407=ORIENTED_EDGE ( 'NONE', *, *, #35118, .F. ) ;
#41408=CARTESIAN_POINT ( 'NONE',  ( -14.59999999999998366, 2.500000000000000000, 0.5928203230275517210 ) ) ;
#41409=ORIENTED_EDGE ( 'NONE', *, *, #29196, .T. ) ;
#41410=DIRECTION ( 'NONE',  ( -0.000000000000000000, 1.000000000000000000, -0.000000000000000000 ) ) ;
#41411=LINE ( 'NONE', #81325, #38741 ) ;
#41412=ADVANCED_FACE ( 'NONE', ( #90604 ), #9128, .T. ) ;
#41413=AXIS2_PLACEMENT_3D ( 'NONE', #25192, #65109, #73645 ) ;
#41414=DIRECTION ( 'NONE',  ( -0.000000000000000000, 1.000000000000000000, -0.000000000000000000 ) ) ;
#41415=VERTEX_POINT ( 'NONE', #40899 ) ;
#41416=ORIENTED_EDGE ( 'NONE', *, *, #71906, .T. ) ;
#41417=FACE_BOUND ( 'NONE', #123490, .T. ) ;
#41418=EDGE_LOOP ( 'NONE', ( #55848, #78269, #78586, #5914 ) ) ;
#41419=EDGE_CURVE ( 'NONE', #36193, #94775, #50902, .T. ) ;
#41420=LINE ( 'NONE', #31584, #34625 ) ;
#41422=CARTESIAN_POINT ( 'NONE',  ( 0.8499999999999545697, 12.50000000000000000, -1.472243186433550122 ) ) ;
#41423=CIRCLE ( 'NONE', #18416, 0.06509327318403745899 ) ;
#41424=FACE_OUTER_BOUND ( 'NONE', #116679, .T. ) ;
#41425=PLANE ( 'NONE',  #112005 ) ;
#41426=DIRECTION ( 'NONE',  ( -0.000000000000000000, -1.000000000000000000, -0.000000000000000000 ) ) ;
#41427=CIRCLE ( 'NONE', #14194, 0.06509327318403745899 ) ;
#41428=DIRECTION ( 'NONE',  ( 0.000000000000000000, 0.000000000000000000, -1.000000000000000000 ) ) ;
#41429=CARTESIAN_POINT ( 'NONE',  ( 9.149999999999920419, 2.500000000000000000, -5.902370205355750521 ) ) ;
#41430=ADVANCED_FACE ( 'NONE', ( #67747 ), #79513, .T. ) ;
#41431=CARTESIAN_POINT ( 'NONE',  ( 1.699999999999951994, 2.500000000000000000, -4.430127018922202176 ) ) ;
#41432=DIRECTION ( 'NONE',  ( 0.000000000000000000, -0.000000000000000000, 1.000000000000000000 ) ) ;
#41433=CIRCLE ( 'NONE', #91583, 0.09999999999999999167 ) ;
#41434=CIRCLE ( 'NONE', #58149, 0.1000000000000000472 ) ;
#41435=DIRECTION ( 'NONE',  ( 0.000000000000000000, 1.000000000000000000, 0.000000000000000000 ) ) ;
#41436=ORIENTED_EDGE ( 'NONE', *, *, #127668, .F. ) ;
#41437=CIRCLE ( 'NONE', #95709, 0.06509327318403745899 ) ;
#41438=ORIENTED_EDGE ( 'NONE', *, *, #70368, .F. ) ;
#41439=VERTEX_POINT ( 'NONE', #70331 ) ;
#41440=ORIENTED_EDGE ( 'NONE', *, *, #119334, .F. ) ;
#41441=LINE ( 'NONE', #51895, #110336 ) ;
#41442=DIRECTION ( 'NONE',  ( -0.000000000000000000, 1.000000000000000000, -0.000000000000000000 ) ) ;
#41443=EDGE_LOOP ( 'NONE', ( #108555, #46555 ) ) ;
#41444=VERTEX_POINT ( 'NONE', #27816 ) ;
#41445=CIRCLE ( 'NONE', #114562, 0.09999999999999999167 ) ;
#41446=ORIENTED_EDGE ( 'NONE', *, *, #123574, .F. ) ;
#41447=PLANE ( 'NONE',  #25042 ) ;
#41448=CARTESIAN_POINT ( 'NONE',  ( 3.349999999999944578, 12.50000000000000000, -5.802370205355749988 ) ) ;
#41449=FILL_AREA_STYLE ('',( #21134 ) ) ;
#41450=CARTESIAN_POINT ( 'NONE',  ( -8.749999999999976907, 2.500000000000000000, -6.495190528383297135 ) ) ;
#41451=DIRECTION ( 'NONE',  ( 0.000000000000000000, 0.000000000000000000, 1.000000000000000000 ) ) ;
#41453=DIRECTION ( 'NONE',  ( -0.000000000000000000, 1.000000000000000000, -0.000000000000000000 ) ) ;
#41454=VECTOR ( 'NONE', #6409, 1000.000000000000000 ) ;
#41455=VERTEX_POINT ( 'NONE', #107679 ) ;
#41456=DIRECTION ( 'NONE',  ( -0.000000000000000000, -1.000000000000000000, -0.000000000000000000 ) ) ;
#41457=ORIENTED_EDGE ( 'NONE', *, *, #29071, .F. ) ;
#41458=ADVANCED_FACE ( 'NONE', ( #17995 ), #48119, .T. ) ;
#41459=CIRCLE ( 'NONE', #123003, 0.06509327318403745899 ) ;
#41460=AXIS2_PLACEMENT_3D ( 'NONE', #72744, #23001, #72105 ) ;
#41461=VERTEX_POINT ( 'NONE', #59241 ) ;
#41462=ORIENTED_EDGE ( 'NONE', *, *, #21227, .F. ) ;
#41463=CARTESIAN_POINT ( 'NONE',  ( 7.899999999999923084, 2.500000000000000000, -0.7928203230275543412 ) ) ;
#41464=ORIENTED_EDGE ( 'NONE', *, *, #78073, .T. ) ;
#41465=EDGE_CURVE ( 'NONE', #89903, #129360, #127956, .T. ) ;
#41466=ORIENTED_EDGE ( 'NONE', *, *, #81890, .T. ) ;
#41467=VERTEX_POINT ( 'NONE', #118134 ) ;
#41468=EDGE_CURVE ( 'NONE', #118944, #81926, #9021, .T. ) ;
#41469=DIRECTION ( 'NONE',  ( -0.000000000000000000, 1.000000000000000000, -0.000000000000000000 ) ) ;
#41471=DIRECTION ( 'NONE',  ( 0.000000000000000000, 0.000000000000000000, 1.000000000000000000 ) ) ;
#41472=PLANE ( 'NONE',  #31606 ) ;
#41473=DIRECTION ( 'NONE',  ( 0.000000000000000000, 0.000000000000000000, 1.000000000000000000 ) ) ;
#41474=EDGE_CURVE ( 'NONE', #86459, #119361, #38300, .T. ) ;
#41475=DIRECTION ( 'NONE',  ( 0.000000000000000000, 0.000000000000000000, -1.000000000000000000 ) ) ;
#41476=EDGE_CURVE ( 'NONE', #76693, #93836, #105274, .T. ) ;
#41477=EDGE_CURVE ( 'NONE', #113011, #110791, #279, .T. ) ;
#41479=EDGE_LOOP ( 'NONE', ( #29574, #35182 ) ) ;
#41480=CIRCLE ( 'NONE', #74908, 0.06509327318403745899 ) ;
#41482=ADVANCED_FACE ( 'NONE', ( #20588 ), #101067, .T. ) ;
#41483=VERTEX_POINT ( 'NONE', #129276 ) ;
#41484=CARTESIAN_POINT ( 'NONE',  ( -7.900000000000014566, 2.500000000000000000, -3.637306695894650055 ) ) ;
#41485=PLANE ( 'NONE',  #12699 ) ;
#41486=CONICAL_SURFACE ( 'NONE', #3800, 0.09999999999999982514, 0.003490658503988666988 ) ;
#41487=AXIS2_PLACEMENT_3D ( 'NONE', #528, #29375, #119034 ) ;
#41488=VERTEX_POINT ( 'NONE', #128635 ) ;
#41489=DIRECTION ( 'NONE',  ( 0.000000000000000000, 1.000000000000000000, 0.000000000000000000 ) ) ;
#41490=ADVANCED_FACE ( 'NONE', ( #60534 ), #44641, .T. ) ;
#41491=VERTEX_POINT ( 'NONE', #29132 ) ;
#41492=ADVANCED_FACE ( 'NONE', ( #69027 ), #108941, .T. ) ;
#41493=CARTESIAN_POINT ( 'NONE',  ( 6.849999999999927702, 12.50000000000000000, 1.818653347947321475 ) ) ;
#41494=CONICAL_SURFACE ( 'NONE', #45677, 0.09999999999999982514, 0.003490658503988666988 ) ;
#41495=AXIS2_PLACEMENT_3D ( 'NONE', #63979, #32618, #81053 ) ;
#41496=PLANE ( 'NONE',  #88581 ) ;
#41497=ORIENTED_EDGE ( 'NONE', *, *, #46912, .T. ) ;
#41498=ORIENTED_EDGE ( 'NONE', *, *, #108825, .F. ) ;
#41499=CARTESIAN_POINT ( 'NONE',  ( -11.25000000000000000, 12.50000000000000000, -2.922977105672687426 ) ) ;
#41500=DIRECTION ( 'NONE',  ( 0.000000000000000000, 0.000000000000000000, 1.000000000000000000 ) ) ;
#41502=FACE_OUTER_BOUND ( 'NONE', #67553, .T. ) ;
#41503=CONICAL_SURFACE ( 'NONE', #24748, 0.09999999999999982514, 0.003490658503988666988 ) ;
#41504=CARTESIAN_POINT ( 'NONE',  ( -4.350000000000023626, 2.500000000000000000, 1.918653347947321564 ) ) ;
#41505=AXIS2_PLACEMENT_3D ( 'NONE', #30102, #88329, #60208 ) ;
#41506=VERTEX_POINT ( 'NONE', #50069 ) ;
#41507=LINE ( 'NONE', #81417, #27852 ) ;
#41508=VERTEX_POINT ( 'NONE', #49416 ) ;
#41509=FACE_OUTER_BOUND ( 'NONE', #29163, .T. ) ;
#41510=DIRECTION ( 'NONE',  ( -0.000000000000000000, 1.000000000000000000, -0.000000000000000000 ) ) ;
#41511=AXIS2_PLACEMENT_3D ( 'NONE', #102092, #113851, #12408 ) ;
#41512=VECTOR ( 'NONE', #76088, 1000.000000000000000 ) ;
#41513=DIRECTION ( 'NONE',  ( 0.000000000000000000, 0.000000000000000000, 1.000000000000000000 ) ) ;
#41514=DIRECTION ( 'NONE',  ( 0.000000000000000000, 1.000000000000000000, 0.000000000000000000 ) ) ;
#41515=DIRECTION ( 'NONE',  ( -0.000000000000000000, 1.000000000000000000, -0.000000000000000000 ) ) ;
#41516=DIRECTION ( 'NONE',  ( 0.000000000000000000, 0.000000000000000000, 1.000000000000000000 ) ) ;
#41517=DIRECTION ( 'NONE',  ( -0.000000000000000000, 1.000000000000000000, -0.000000000000000000 ) ) ;
#41518=VERTEX_POINT ( 'NONE', #89328 ) ;
#41519=CONICAL_SURFACE ( 'NONE', #70741, 0.1000000000000002554, 0.003490658503988666988 ) ;
#41520=DIRECTION ( 'NONE',  ( 0.000000000000000000, -0.9999939076577903929, 0.003490651415223739937 ) ) ;
#41521=EDGE_CURVE ( 'NONE', #17072, #121453, #39609, .T. ) ;
#41523=CARTESIAN_POINT ( 'NONE',  ( 1.049999999999954081, 2.500000000000000000, -6.048780366869526581 ) ) ;
#41525=ADVANCED_FACE ( 'NONE', ( #19948 ), #59891, .T. ) ;
#41526=EDGE_LOOP ( 'NONE', ( #64552, #92627 ) ) ;
#41527=AXIS2_PLACEMENT_3D ( 'NONE', #109705, #20034, #61900 ) ;
#41528=CARTESIAN_POINT ( 'NONE',  ( -3.750000000000025757, 12.50000000000000000, 1.472243186433545459 ) ) ;
#41529=VECTOR ( 'NONE', #125050, 1000.000000000000000 ) ;
#41530=ORIENTED_EDGE ( 'NONE', *, *, #60670, .T. ) ;
#41531=ORIENTED_EDGE ( 'NONE', *, *, #128347, .F. ) ;
#41532=CARTESIAN_POINT ( 'NONE',  ( -7.700000000000010836, 2.500000000000000000, 3.983716857408420964 ) ) ;
#41533=EDGE_LOOP ( 'NONE', ( #2603, #120466, #4076, #89880 ) ) ;
#41534=CARTESIAN_POINT ( 'NONE',  ( 8.099999999999923261, 12.50000000000000000, -4.741630453620016006 ) ) ;
#41535=AXIS2_PLACEMENT_3D ( 'NONE', #42718, #123192, #2102 ) ;
#41536=CARTESIAN_POINT ( 'NONE',  ( 3.149999999999942624, 12.50000000000000000, 6.148780366869520897 ) ) ;
#41537=VERTEX_POINT ( 'NONE', #73535 ) ;
#41538=DIRECTION ( 'NONE',  ( -0.000000000000000000, 1.000000000000000000, -0.000000000000000000 ) ) ;
#41539=DIRECTION ( 'NONE',  ( 0.000000000000000000, 1.000000000000000000, 0.000000000000000000 ) ) ;
#41540=CONICAL_SURFACE ( 'NONE', #70762, 0.1000000000000002554, 0.003490658503988666988 ) ;
#41541=EDGE_LOOP ( 'NONE', ( #122341, #39 ) ) ;
#41542=AXIS2_PLACEMENT_3D ( 'NONE', #112500, #22846, #102662 ) ;
#41543=ORIENTED_EDGE ( 'NONE', *, *, #109089, .T. ) ;
#41544=ORIENTED_EDGE ( 'NONE', *, *, #103804, .T. ) ;
#41545=PLANE ( 'NONE',  #75553 ) ;
#41546=DIRECTION ( 'NONE',  ( 0.000000000000000000, 0.000000000000000000, 1.000000000000000000 ) ) ;
#41547=CARTESIAN_POINT ( 'NONE',  ( 8.149999999999923972, 2.500000000000000000, -6.841600689897077814 ) ) ;
#41548=FACE_BOUND ( 'NONE', #48550, .T. ) ;
#41549=ORIENTED_EDGE ( 'NONE', *, *, #81773, .F. ) ;
#41550=DIRECTION ( 'NONE',  ( 0.000000000000000000, 0.000000000000000000, -1.000000000000000000 ) ) ;
#41551=FACE_OUTER_BOUND ( 'NONE', #37449, .T. ) ;
#41552=EDGE_LOOP ( 'NONE', ( #95032, #35077 ) ) ;
#41553=DIRECTION ( 'NONE',  ( 0.000000000000000000, 1.000000000000000000, 0.000000000000000000 ) ) ;
#41554=EDGE_CURVE ( 'NONE', #42734, #14735, #65458, .T. ) ;
#41555=CARTESIAN_POINT ( 'NONE',  ( -4.600000000000025402, 12.50000000000000000, 4.330127018922196314 ) ) ;
#41556=CARTESIAN_POINT ( 'NONE',  ( -10.45000000000000462, 12.50000000000000000, -2.165063509461097713 ) ) ;
#41557=CARTESIAN_POINT ( 'NONE',  ( 4.149999999999939959, 12.50000000000000000, -2.165063509461101710 ) ) ;
#41558=CIRCLE ( 'NONE', #66566, 0.09999999999999982514 ) ;
#41559=DIRECTION ( 'NONE',  ( 0.000000000000000000, 0.000000000000000000, 1.000000000000000000 ) ) ;
#41560=DIRECTION ( 'NONE',  ( 0.000000000000000000, 0.000000000000000000, 1.000000000000000000 ) ) ;
#41561=CARTESIAN_POINT ( 'NONE',  ( 1.049999999999952083, 2.500000000000000000, 6.941600689897073018 ) ) ;
#41562=EDGE_CURVE ( 'NONE', #42779, #31532, #15366, .T. ) ;
#41563=AXIS2_PLACEMENT_3D ( 'NONE', #34744, #104726, #106038 ) ;
#41564=CIRCLE ( 'NONE', #114694, 0.09999999999999982514 ) ;
#41565=EDGE_LOOP ( 'NONE', ( #101866, #29712 ) ) ;
#41566=ORIENTED_EDGE ( 'NONE', *, *, #57148, .F. ) ;
#41567=CONICAL_SURFACE ( 'NONE', #58282, 0.1000000000000002554, 0.003490658503988666988 ) ;
#41568=ORIENTED_EDGE ( 'NONE', *, *, #11190, .F. ) ;
#41569=ORIENTED_EDGE ( 'NONE', *, *, #116970, .T. ) ;
#41570=DIRECTION ( 'NONE',  ( 0.000000000000000000, -0.000000000000000000, 1.000000000000000000 ) ) ;
#41571=ADVANCED_FACE ( 'NONE', ( #22541 ), #31700, .T. ) ;
#41572=LINE ( 'NONE', #81480, #92769 ) ;
#41573=EDGE_LOOP ( 'NONE', ( #114302, #12106 ) ) ;
#41574=FACE_BOUND ( 'NONE', #24451, .T. ) ;
#41575=EDGE_CURVE ( 'NONE', #126915, #65424, #98920, .T. ) ;
#41576=PLANE ( 'NONE',  #58460 ) ;
#41577=DIRECTION ( 'NONE',  ( -0.000000000000000000, -1.000000000000000000, -0.000000000000000000 ) ) ;
#41578=AXIS2_PLACEMENT_3D ( 'NONE', #45941, #17069, #126428 ) ;
#41579=VECTOR ( 'NONE', #45647, 1000.000000000000000 ) ;
#41580=CARTESIAN_POINT ( 'NONE',  ( -13.34999999999999076, 12.50000000000000000, -1.407149913249510442 ) ) ;
#41581=CIRCLE ( 'NONE', #18572, 0.1000000000000000056 ) ;
#41582=EDGE_CURVE ( 'NONE', #97417, #73329, #78085, .T. ) ;
#41583=DIRECTION ( 'NONE',  ( 0.000000000000000000, 0.000000000000000000, -1.000000000000000000 ) ) ;
#41584=FACE_OUTER_BOUND ( 'NONE', #93337, .T. ) ;
#41585=CARTESIAN_POINT ( 'NONE',  ( -1.250000000000001554, 12.50000000000000000, 6.430097255199259010 ) ) ;
#41586=DIRECTION ( 'NONE',  ( -0.000000000000000000, 1.000000000000000000, -0.000000000000000000 ) ) ;
#41587=FACE_OUTER_BOUND ( 'NONE', #16317, .T. ) ;
#41588=EDGE_CURVE ( 'NONE', #102089, #5504, #112837, .T. ) ;
#41589=DIRECTION ( 'NONE',  ( -4.274815082592931898E-19, -0.9999939076577903929, -0.003490651415223739937 ) ) ;
#41590=VERTEX_POINT ( 'NONE', #63084 ) ;
#41591=AXIS2_PLACEMENT_3D ( 'NONE', #126022, #24623, #23980 ) ;
#41592=VERTEX_POINT ( 'NONE', #51358 ) ;
#41593=CONICAL_SURFACE ( 'NONE', #10178, 0.1000000000000000472, 0.003490658503988666988 ) ;
#41595=VERTEX_POINT ( 'NONE', #91258 ) ;
#41596=ORIENTED_EDGE ( 'NONE', *, *, #88687, .T. ) ;
#41597=ORIENTED_EDGE ( 'NONE', *, *, #14376, .F. ) ;
#41598=CARTESIAN_POINT ( 'NONE',  ( -0.2000000000000399791, 2.500000000000000000, -4.576537180435977348 ) ) ;
#41600=DIRECTION ( 'NONE',  ( -0.000000000000000000, -1.000000000000000000, -0.000000000000000000 ) ) ;
#41601=CARTESIAN_POINT ( 'NONE',  ( 1.849999999999950573, 12.50000000000000000, -1.818653347947326138 ) ) ;
#41602=FACE_OUTER_BOUND ( 'NONE', #99840, .T. ) ;
#41603=DIRECTION ( 'NONE',  ( 0.000000000000000000, 0.000000000000000000, -1.000000000000000000 ) ) ;
#41604=CIRCLE ( 'NONE', #22725, 0.09999999999999999167 ) ;
#41605=ORIENTED_EDGE ( 'NONE', *, *, #91198, .T. ) ;
#41606=CARTESIAN_POINT ( 'NONE',  ( 3.749999999999976907, 2.500000000000000000, 2.165063509461097713 ) ) ;
#41607=ORIENTED_EDGE ( 'NONE', *, *, #3846, .T. ) ;
#41608=EDGE_CURVE ( 'NONE', #43343, #24753, #55105, .T. ) ;
#41609=EDGE_LOOP ( 'NONE', ( #37173, #4746 ) ) ;
#41610=VECTOR ( 'NONE', #109724, 1000.000000000000000 ) ;
#41611=DIRECTION ( 'NONE',  ( 0.000000000000000000, 0.000000000000000000, 1.000000000000000000 ) ) ;
#41612=DIRECTION ( 'NONE',  ( 0.000000000000000000, 1.000000000000000000, 0.000000000000000000 ) ) ;
#41613=DIRECTION ( 'NONE',  ( 0.000000000000000000, 0.000000000000000000, -1.000000000000000000 ) ) ;
#41614=EDGE_CURVE ( 'NONE', #74146, #13780, #75927, .T. ) ;
#41615=VERTEX_POINT ( 'NONE', #12678 ) ;
#41616=CONICAL_SURFACE ( 'NONE', #37402, 0.09999999999999982514, 0.003490658503988666988 ) ;
#41617=ORIENTED_EDGE ( 'NONE', *, *, #124628, .F. ) ;
#41618=EDGE_CURVE ( 'NONE', #110642, #46368, #36236, .T. ) ;
#41619=DIRECTION ( 'NONE',  ( 0.000000000000000000, 0.000000000000000000, 1.000000000000000000 ) ) ;
#41620=VECTOR ( 'NONE', #128947, 1000.000000000000000 ) ;
#41621=DIRECTION ( 'NONE',  ( 0.000000000000000000, -0.000000000000000000, 1.000000000000000000 ) ) ;
#41622=LINE ( 'NONE', #120163, #95785 ) ;
#41623=DIRECTION ( 'NONE',  ( 0.000000000000000000, -0.9999939076577903929, 0.003490651415223739937 ) ) ;
#41624=EDGE_LOOP ( 'NONE', ( #32368, #91331, #127727, #9638 ) ) ;
#41625=ADVANCED_FACE ( 'NONE', ( #103001 ), #32139, .T. ) ;
#41626=ADVANCED_FACE ( 'NONE', ( #13326 ), #86388, .T. ) ;
#41627=DIRECTION ( 'NONE',  ( -0.000000000000000000, -1.000000000000000000, -0.000000000000000000 ) ) ;
#41628=AXIS2_PLACEMENT_3D ( 'NONE', #61881, #50129, #100492 ) ;
#41629=ADVANCED_FACE ( 'NONE', ( #91904 ), #96850, .T. ) ;
#41630=EDGE_CURVE ( 'NONE', #8036, #52810, #6948, .T. ) ;
#41631=ORIENTED_EDGE ( 'NONE', *, *, #41875, .T. ) ;
#41632=CARTESIAN_POINT ( 'NONE',  ( 14.69113575804714422, -2.499999999999999556, 6.337000356225073183 ) ) ;
#41634=DIRECTION ( 'NONE',  ( 0.000000000000000000, 0.000000000000000000, 1.000000000000000000 ) ) ;
#41635=CIRCLE ( 'NONE', #22849, 0.09999999999999999167 ) ;
#41636=CONICAL_SURFACE ( 'NONE', #75059, 0.1000000000000000056, 0.003490658503988666988 ) ;
#41637=EDGE_CURVE ( 'NONE', #54383, #91134, #9222, .T. ) ;
#41638=DIRECTION ( 'NONE',  ( -0.000000000000000000, 1.000000000000000000, -0.000000000000000000 ) ) ;
#41639=CARTESIAN_POINT ( 'NONE',  ( -2.500000000000032419, 12.50000000000000000, 0.6277270498435120194 ) ) ;
#41640=CONICAL_SURFACE ( 'NONE', #129471, 0.1000000000000000056, 0.003490658503988666988 ) ;
#41641=LINE ( 'NONE', #103106, #94711 ) ;
#41642=FACE_OUTER_BOUND ( 'NONE', #122117, .T. ) ;
#41643=ORIENTED_EDGE ( 'NONE', *, *, #45021, .T. ) ;
#41644=ADVANCED_FACE ( 'NONE', ( #3523 ), #2869, .T. ) ;
#41645=DIRECTION ( 'NONE',  ( 0.000000000000000000, 0.000000000000000000, -1.000000000000000000 ) ) ;
#41646=CONICAL_SURFACE ( 'NONE', #106454, 0.1000000000000002554, 0.003490658503988666988 ) ;
#41647=AXIS2_PLACEMENT_3D ( 'NONE', #88825, #89475, #30577 ) ;
#41648=EDGE_CURVE ( 'NONE', #91650, #110814, #33633, .T. ) ;
#41649=CARTESIAN_POINT ( 'NONE',  ( 2.299999999999949640, 12.50000000000000000, -4.611443907251939756 ) ) ;
#41650=ORIENTED_EDGE ( 'NONE', *, *, #10836, .T. ) ;
#41651=ORIENTED_EDGE ( 'NONE', *, *, #44869, .F. ) ;
#41652=ORIENTED_EDGE ( 'NONE', *, *, #81640, .F. ) ;
#41653=CARTESIAN_POINT ( 'NONE',  ( 17.50000000000000000, -2.750000000000000000, 10.00000000000000178 ) ) ;
#41654=CARTESIAN_POINT ( 'NONE',  ( 14.14999999999989377, 12.50000000000000000, -1.472243186433550122 ) ) ;
#41655=DIRECTION ( 'NONE',  ( -4.274815082592931898E-19, -0.9999939076577903929, -0.003490651415223739937 ) ) ;
#41656=LINE ( 'NONE', #2322, #92520 ) ;
#41657=DIRECTION ( 'NONE',  ( 0.000000000000000000, 0.000000000000000000, -1.000000000000000000 ) ) ;
#41658=CARTESIAN_POINT ( 'NONE',  ( 7.499999999999927169, 12.50000000000000000, 3.572213422710607489 ) ) ;
#41659=CARTESIAN_POINT ( 'NONE',  ( -3.100000000000028511, 12.50000000000000000, 0.4115034346978110880 ) ) ;
#41660=VECTOR ( 'NONE', #22885, 1000.000000000000000 ) ;
#41661=AXIS2_PLACEMENT_3D ( 'NONE', #125514, #65951, #56750 ) ;
#41662=CONICAL_SURFACE ( 'NONE', #6111, 0.09999999999999999167, 0.003490658503988666988 ) ;
#41663=VERTEX_POINT ( 'NONE', #63739 ) ;
#41664=CARTESIAN_POINT ( 'NONE',  ( 5.799999999999933209, 2.500000000000000000, -0.1000000000000023925 ) ) ;
#41665=CARTESIAN_POINT ( 'NONE',  ( 2.049999999999948308, 12.50000000000000000, 6.495190528383297135 ) ) ;
#41666=CARTESIAN_POINT ( 'NONE',  ( -7.700000000000014388, 2.500000000000000000, -4.576537180435977348 ) ) ;
#41667=CARTESIAN_POINT ( 'NONE',  ( 0.8499999999999536815, 12.50000000000000000, 5.802370205355744659 ) ) ;
#41668=CIRCLE ( 'NONE', #106385, 0.1000000000000002554 ) ;
#41669=VERTEX_POINT ( 'NONE', #104920 ) ;
#41670=AXIS2_PLACEMENT_3D ( 'NONE', #28574, #58682, #126778 ) ;
#41671=CARTESIAN_POINT ( 'NONE',  ( 5.849999999999931255, 2.500000000000000000, 2.857883832488649301 ) ) ;
#41672=CONICAL_SURFACE ( 'NONE', #100234, 0.09999999999999982514, 0.003490658503988666988 ) ;
#41673=EDGE_CURVE ( 'NONE', #52514, #22700, #94902, .T. ) ;
#41674=DIRECTION ( 'NONE',  ( 0.000000000000000000, -0.000000000000000000, 1.000000000000000000 ) ) ;
#41675=CARTESIAN_POINT ( 'NONE',  ( 0.3999999999999568345, 2.500000000000000000, -3.737306695894649700 ) ) ;
#41676=EDGE_LOOP ( 'NONE', ( #5514, #55283, #57668, #63483 ) ) ;
#41677=VECTOR ( 'NONE', #34299, 1000.000000000000000 ) ;
#41678=ORIENTED_EDGE ( 'NONE', *, *, #28941, .T. ) ;
#41679=CARTESIAN_POINT ( 'NONE',  ( 9.799999999999915445, 2.500000000000000000, -4.576537180435977348 ) ) ;
#41680=EDGE_CURVE ( 'NONE', #21282, #105322, #117872, .T. ) ;
#41681=CONICAL_SURFACE ( 'NONE', #8195, 0.1000000000000000472, 0.003490658503988666988 ) ;
#41682=ORIENTED_EDGE ( 'NONE', *, *, #95815, .T. ) ;
#41683=ORIENTED_EDGE ( 'NONE', *, *, #33932, .T. ) ;
#41684=DIRECTION ( 'NONE',  ( -0.000000000000000000, -1.000000000000000000, -0.000000000000000000 ) ) ;
#41685=DIRECTION ( 'NONE',  ( -0.000000000000000000, -1.000000000000000000, -0.000000000000000000 ) ) ;
#41686=DIRECTION ( 'NONE',  ( 0.000000000000000000, 0.000000000000000000, -1.000000000000000000 ) ) ;
#41687=CARTESIAN_POINT ( 'NONE',  ( -14.34999999999998543, 2.500000000000000000, 2.611473670974877148 ) ) ;
#41688=EDGE_LOOP ( 'NONE', ( #60749, #115168, #14230, #16436 ) ) ;
#41689=CARTESIAN_POINT ( 'NONE',  ( -8.950000000000004619, 2.500000000000000000, 6.148780366869520897 ) ) ;
#41690=ORIENTED_EDGE ( 'NONE', *, *, #18403, .T. ) ;
#41691=CARTESIAN_POINT ( 'NONE',  ( -9.150000000000009237, 12.50000000000000000, 2.099970236277060032 ) ) ;
#41694=ORIENTED_EDGE ( 'NONE', *, *, #77731, .F. ) ;
#41696=ORIENTED_EDGE ( 'NONE', *, *, #16355, .T. ) ;
#41697=PLANE ( 'NONE',  #69199 ) ;
#41698=CARTESIAN_POINT ( 'NONE',  ( 6.714630671504235870, 2.500000000000252687, 9.763603585389109440 ) ) ;
#41699=CARTESIAN_POINT ( 'NONE',  ( 13.94999999999989626, 2.500000000000000000, 2.511473670974873507 ) ) ;
#41700=FACE_BOUND ( 'NONE', #51622, .T. ) ;
#41701=VERTEX_POINT ( 'NONE', #125858 ) ;
#41702=CARTESIAN_POINT ( 'NONE',  ( 11.89999999999990798, 2.500000000000000000, 4.676537180435972552 ) ) ;
#41704=AXIS2_PLACEMENT_3D ( 'NONE', #107450, #96985, #104857 ) ;
#41705=DIRECTION ( 'NONE',  ( -0.000000000000000000, -1.000000000000000000, -0.000000000000000000 ) ) ;
#41706=DIRECTION ( 'NONE',  ( -4.274815082592931898E-19, -0.9999939076577903929, -0.003490651415223739937 ) ) ;
#41707=PLANE ( 'NONE',  #86125 ) ;
#41708=CARTESIAN_POINT ( 'NONE',  ( 13.74999999999989342, 2.500000000000000000, -1.472243186433550122 ) ) ;
#41709=CIRCLE ( 'NONE', #47962, 0.06509327318403745899 ) ;
#41710=CARTESIAN_POINT ( 'NONE',  ( 4.799999999999934097, 2.500000000000000000, 4.676537180435972552 ) ) ;
#41711=ADVANCED_FACE ( 'NONE', ( #116687 ), #115374, .T. ) ;
#41712=LINE ( 'NONE', #12220, #3453 ) ;
#41713=CIRCLE ( 'NONE', #24967, 0.06509327318403741736 ) ;
#41714=CONICAL_SURFACE ( 'NONE', #114842, 0.1000000000000000056, 0.003490658503988666988 ) ;
#41715=VERTEX_POINT ( 'NONE', #25091 ) ;
#41716=VERTEX_POINT ( 'NONE', #84000 ) ;
#41717=ORIENTED_EDGE ( 'NONE', *, *, #105110, .T. ) ;
#41718=ORIENTED_EDGE ( 'NONE', *, *, #17921, .T. ) ;
#41719=EDGE_LOOP ( 'NONE', ( #43520, #36097, #29287, #65461 ) ) ;
#41720=CARTESIAN_POINT ( 'NONE',  ( -6.250000000000017764, 12.50000000000000000, 7.188010851410848723 ) ) ;
#41721=CIRCLE ( 'NONE', #68877, 0.1000000000000002554 ) ;
#41722=EDGE_CURVE ( 'NONE', #14537, #93110, #95132, .T. ) ;
#41723=ADVANCED_FACE ( 'NONE', ( #56471 ), #42602, .T. ) ;
#41724=CARTESIAN_POINT ( 'NONE',  ( 10.39999999999991154, 2.500000000000000000, 5.122947341949749323 ) ) ;
#41725=VERTEX_POINT ( 'NONE', #104301 ) ;
#41726=FACE_BOUND ( 'NONE', #87126, .T. ) ;
#41727=ADVANCED_FACE ( 'NONE', ( #74845 ), #99011, .T. ) ;
#41728=CARTESIAN_POINT ( 'NONE',  ( -13.34999999999999076, 12.50000000000000000, -1.472243186433547901 ) ) ;
#41729=AXIS2_PLACEMENT_3D ( 'NONE', #77669, #8284, #106498 ) ;
#41730=VECTOR ( 'NONE', #30902, 1000.000000000000000 ) ;
#41731=ADVANCED_FACE ( 'NONE', ( #85927 ), #109476, .T. ) ;
#41732=ORIENTED_EDGE ( 'NONE', *, *, #10129, .T. ) ;
#41733=DIRECTION ( 'NONE',  ( -0.000000000000000000, -1.000000000000000000, -0.000000000000000000 ) ) ;
#41734=CARTESIAN_POINT ( 'NONE',  ( -2.499999999999996447, 2.500000000000000000, 4.330127018922196314 ) ) ;
#41735=PLANE ( 'NONE',  #9290 ) ;
#41736=ADVANCED_FACE ( 'NONE', ( #17169 ), #78190, .T. ) ;
#41737=CARTESIAN_POINT ( 'NONE',  ( -6.850000000000013856, 2.500000000000000000, 6.841600689897072485 ) ) ;
#41738=ORIENTED_EDGE ( 'NONE', *, *, #84332, .T. ) ;
#41739=CARTESIAN_POINT ( 'NONE',  ( -3.749999999999994671, 12.50000000000000000, -6.495190528383302464 ) ) ;
#41740=ORIENTED_EDGE ( 'NONE', *, *, #120648, .T. ) ;
#41741=ORIENTED_EDGE ( 'NONE', *, *, #53824, .T. ) ;
#41742=ORIENTED_EDGE ( 'NONE', *, *, #90947, .F. ) ;
#41743=CONICAL_SURFACE ( 'NONE', #70965, 0.09999999999999999167, 0.003490658503988666988 ) ;
#41744=DIRECTION ( 'NONE',  ( 0.000000000000000000, 0.000000000000000000, 1.000000000000000000 ) ) ;
#41745=DIRECTION ( 'NONE',  ( 0.000000000000000000, 1.000000000000000000, 0.000000000000000000 ) ) ;
#41746=EDGE_LOOP ( 'NONE', ( #106018, #20745 ) ) ;
#41747=DIRECTION ( 'NONE',  ( -0.000000000000000000, 1.000000000000000000, -0.000000000000000000 ) ) ;
#41748=AXIS2_PLACEMENT_3D ( 'NONE', #42142, #34272, #2858 ) ;
#41749=DIRECTION ( 'NONE',  ( 0.000000000000000000, 0.000000000000000000, 1.000000000000000000 ) ) ;
#41750=DIRECTION ( 'NONE',  ( -0.000000000000000000, 1.000000000000000000, -0.000000000000000000 ) ) ;
#41751=DIRECTION ( 'NONE',  ( -0.000000000000000000, 1.000000000000000000, -0.000000000000000000 ) ) ;
#41753=ORIENTED_EDGE ( 'NONE', *, *, #99502, .F. ) ;
#41754=CARTESIAN_POINT ( 'NONE',  ( 2.899999999999946620, 2.500000000000000000, 0.5928203230275495006 ) ) ;
#41755=AXIS2_PLACEMENT_3D ( 'NONE', #15867, #55805, #26999 ) ;
#41756=EDGE_LOOP ( 'NONE', ( #89868, #13320, #117603, #40161 ) ) ;
#41757=DIRECTION ( 'NONE',  ( -0.000000000000000000, -1.000000000000000000, -0.000000000000000000 ) ) ;
#41758=AXIS2_PLACEMENT_3D ( 'NONE', #58354, #9240, #28237 ) ;
#41759=AXIS2_PLACEMENT_3D ( 'NONE', #36623, #66695, #85692 ) ;
#41760=VERTEX_POINT ( 'NONE', #27032 ) ;
#41761=DIRECTION ( 'NONE',  ( 0.000000000000000000, -0.9999939076577903929, 0.003490651415223739937 ) ) ;
#41762=ORIENTED_EDGE ( 'NONE', *, *, #46585, .T. ) ;
#41763=DIRECTION ( 'NONE',  ( -0.000000000000000000, 1.000000000000000000, -0.000000000000000000 ) ) ;
#41765=CARTESIAN_POINT ( 'NONE',  ( 0.6499999999999566125, 2.500000000000000000, -6.048780366869526581 ) ) ;
#41766=DIRECTION ( 'NONE',  ( -0.000000000000000000, -1.000000000000000000, -0.000000000000000000 ) ) ;
#41767=CARTESIAN_POINT ( 'NONE',  ( 97.50000000000000000, 0.000000000000000000, 7.500000000000000000 ) ) ;
#41768=AXIS2_PLACEMENT_3D ( 'NONE', #83861, #15095, #53765 ) ;
#41769=ORIENTED_EDGE ( 'NONE', *, *, #37633, .F. ) ;
#41770=ORIENTED_EDGE ( 'NONE', *, *, #125528, .T. ) ;
#41771=CONICAL_SURFACE ( 'NONE', #45871, 0.1000000000000000472, 0.003490658503988666988 ) ;
#41772=ORIENTED_EDGE ( 'NONE', *, *, #76925, .F. ) ;
#41773=CARTESIAN_POINT ( 'NONE',  ( -8.550000000000011369, 12.50000000000000000, -2.511473670974877948 ) ) ;
#41774=AXIS2_PLACEMENT_3D ( 'NONE', #95125, #16532, #114746 ) ;
#41775=DIRECTION ( 'NONE',  ( -0.000000000000000000, -1.000000000000000000, -0.000000000000000000 ) ) ;
#41776=CARTESIAN_POINT ( 'NONE',  ( -13.54999999999999005, 2.500000000000000000, -1.818653347947323917 ) ) ;
#41777=EDGE_CURVE ( 'NONE', #121648, #34168, #115727, .T. ) ;
#41778=ORIENTED_EDGE ( 'NONE', *, *, #94823, .T. ) ;
#41779=VERTEX_POINT ( 'NONE', #36218 ) ;
#41780=EDGE_LOOP ( 'NONE', ( #45071, #112328, #53891, #53759 ) ) ;
#41781=EDGE_CURVE ( 'NONE', #115124, #65093, #103216, .T. ) ;
#41782=DIRECTION ( 'NONE',  ( 0.000000000000000000, 1.000000000000000000, 0.000000000000000000 ) ) ;
#41783=EDGE_CURVE ( 'NONE', #35444, #90867, #111629, .T. ) ;
#41784=ORIENTED_EDGE ( 'NONE', *, *, #7789, .T. ) ;
#41785=CARTESIAN_POINT ( 'NONE',  ( -0.4500000000000397571, 12.50000000000000000, -6.495190528383302464 ) ) ;
#41786=CARTESIAN_POINT ( 'NONE',  ( -0.2000000000000408673, 12.50000000000000000, -3.983716857408426293 ) ) ;
#41787=CARTESIAN_POINT ( 'NONE',  ( 1.849999999999951017, 2.500000000000000000, -6.048780366869526581 ) ) ;
#41788=DIRECTION ( 'NONE',  ( -4.274815082592931898E-19, -0.9999939076577903929, -0.003490651415223739937 ) ) ;
#41789=DIRECTION ( 'NONE',  ( -4.274815082592931898E-19, -0.9999939076577903929, -0.003490651415223739937 ) ) ;
#41790=EDGE_CURVE ( 'NONE', #77714, #113705, #17522, .T. ) ;
#41791=CARTESIAN_POINT ( 'NONE',  ( 14.59999999999989484, 2.500000000000000000, -0.1000000000000022815 ) ) ;
#41792=DIRECTION ( 'NONE',  ( 0.000000000000000000, 0.000000000000000000, 1.000000000000000000 ) ) ;
#41793=DIRECTION ( 'NONE',  ( 0.000000000000000000, 1.000000000000000000, 0.000000000000000000 ) ) ;
#41794=ORIENTED_EDGE ( 'NONE', *, *, #99872, .T. ) ;
#41795=EDGE_CURVE ( 'NONE', #3331, #12469, #6704, .T. ) ;
#41796=DIRECTION ( 'NONE',  ( -0.000000000000000000, 1.000000000000000000, -0.000000000000000000 ) ) ;
#41797=EDGE_CURVE ( 'NONE', #106728, #27665, #90697, .T. ) ;
#41798=CARTESIAN_POINT ( 'NONE',  ( 35.03103265464613969, -3.271231620382011762, 3.345711933271832361 ) ) ;
#41799=ORIENTED_EDGE ( 'NONE', *, *, #71010, .F. ) ;
#41800=( BOUNDED_CURVE ( )  B_SPLINE_CURVE ( 2, ( #34908, #104270, #103632 ),
 .UNSPECIFIED., .F., .F. ) 
 B_SPLINE_CURVE_WITH_KNOTS ( ( 3, 3 ),
 ( 0.000000000000000000, 8.005299705393619772E-05 ),
 .UNSPECIFIED. ) 
 CURVE ( )  GEOMETRIC_REPRESENTATION_ITEM ( )  RATIONAL_B_SPLINE_CURVE ( ( 1.000000000000000000, 0.9972072019273716670, 0.9944676636816938142 ) ) 
 REPRESENTATION_ITEM ( '' )  );
#41801=ORIENTED_EDGE ( 'NONE', *, *, #17164, .T. ) ;
#41803=DIRECTION ( 'NONE',  ( 0.000000000000000000, 0.000000000000000000, -1.000000000000000000 ) ) ;
#41804=CARTESIAN_POINT ( 'NONE',  ( -10.85000000000000142, 12.50000000000000000, -5.867463478539783672 ) ) ;
#41806=DIRECTION ( 'NONE',  ( 0.000000000000000000, 1.000000000000000000, 0.000000000000000000 ) ) ;
#41807=CARTESIAN_POINT ( 'NONE',  ( 0.7999999999999612976, 2.500000000000000000, -1.084202172485504434E-16 ) ) ;
#41808=DIRECTION ( 'NONE',  ( 0.000000000000000000, 1.000000000000000000, 0.000000000000000000 ) ) ;
#41809=DIRECTION ( 'NONE',  ( -0.000000000000000000, -1.000000000000000000, -0.000000000000000000 ) ) ;
#41810=DIRECTION ( 'NONE',  ( 0.000000000000000000, 1.000000000000000000, 0.000000000000000000 ) ) ;
#41811=AXIS2_PLACEMENT_3D ( 'NONE', #107266, #4524, #26776 ) ;
#41812=DIRECTION ( 'NONE',  ( 0.000000000000000000, 1.000000000000000000, 0.000000000000000000 ) ) ;
#41813=ORIENTED_EDGE ( 'NONE', *, *, #77801, .T. ) ;
#41814=ORIENTED_EDGE ( 'NONE', *, *, #35834, .T. ) ;
#41815=AXIS2_PLACEMENT_3D ( 'NONE', #112959, #105723, #23945 ) ;
#41816=ORIENTED_EDGE ( 'NONE', *, *, #48690, .F. ) ;
#41817=EDGE_LOOP ( 'NONE', ( #90099, #51532 ) ) ;
#41819=DIRECTION ( 'NONE',  ( 0.000000000000000000, 1.000000000000000000, 0.000000000000000000 ) ) ;
#41820=VECTOR ( 'NONE', #110843, 1000.000000000000000 ) ;
#41821=AXIS2_PLACEMENT_3D ( 'NONE', #86412, #17676, #78562 ) ;
#41822=VERTEX_POINT ( 'NONE', #35569 ) ;
#41823=DIRECTION ( 'NONE',  ( 0.000000000000000000, 1.000000000000000000, 0.000000000000000000 ) ) ;
#41824=LINE ( 'NONE', #90236, #11197 ) ;
#41825=DIRECTION ( 'NONE',  ( 0.000000000000000000, 1.000000000000000000, 0.000000000000000000 ) ) ;
#41826=DIRECTION ( 'NONE',  ( 0.000000000000000000, 0.000000000000000000, 1.000000000000000000 ) ) ;
#41827=VERTEX_POINT ( 'NONE', #49264 ) ;
#41828=DIRECTION ( 'NONE',  ( -4.274815082592931898E-19, -0.9999939076577903929, -0.003490651415223739937 ) ) ;
#41829=CARTESIAN_POINT ( 'NONE',  ( -7.500000000000015099, 12.50000000000000000, -5.022947341949754119 ) ) ;
#41831=ADVANCED_FACE ( 'NONE', ( #98330 ), #60379, .T. ) ;
#41832=ORIENTED_EDGE ( 'NONE', *, *, #44549, .F. ) ;
#41833=ORIENTED_EDGE ( 'NONE', *, *, #72633, .T. ) ;
#41834=EDGE_LOOP ( 'NONE', ( #36303, #128132, #48189, #18026 ) ) ;
#41835=DIRECTION ( 'NONE',  ( 0.000000000000000000, 0.000000000000000000, -1.000000000000000000 ) ) ;
#41836=DIRECTION ( 'NONE',  ( 0.000000000000000000, 1.000000000000000000, 0.000000000000000000 ) ) ;
#41837=DIRECTION ( 'NONE',  ( 0.000000000000000000, 1.000000000000000000, 0.000000000000000000 ) ) ;
#41838=CONICAL_SURFACE ( 'NONE', #35568, 0.09999999999999999167, 0.003490658503988666988 ) ;
#41839=EDGE_LOOP ( 'NONE', ( #61134, #5996, #107416, #118987 ) ) ;
#41840=CONICAL_SURFACE ( 'NONE', #112922, 0.1000000000000002554, 0.003490658503988666988 ) ;
#41841=CARTESIAN_POINT ( 'NONE',  ( 13.34999999999990017, 12.50000000000000000, 2.922977105672686982 ) ) ;
#41842=ORIENTED_EDGE ( 'NONE', *, *, #103478, .F. ) ;
#41843=DIRECTION ( 'NONE',  ( -0.000000000000000000, -1.000000000000000000, -0.000000000000000000 ) ) ;
#41844=DIRECTION ( 'NONE',  ( 0.000000000000000000, 0.000000000000000000, 1.000000000000000000 ) ) ;
#41845=CARTESIAN_POINT ( 'NONE',  ( 1.249999999999988454, 2.500000000000000000, 2.165063509461097713 ) ) ;
#41846=CARTESIAN_POINT ( 'NONE',  ( -1.850000000000033840, 12.50000000000000000, 1.818653347947321475 ) ) ;
#41847=VECTOR ( 'NONE', #45698, 1000.000000000000000 ) ;
#41848=ORIENTED_EDGE ( 'NONE', *, *, #41003, .F. ) ;
#41849=ORIENTED_EDGE ( 'NONE', *, *, #101906, .T. ) ;
#41850=ORIENTED_EDGE ( 'NONE', *, *, #74734, .F. ) ;
#41851=CARTESIAN_POINT ( 'NONE',  ( -1.900000000000034994, 2.500000000000000000, -0.2464101615137783419 ) ) ;
#41852=LINE ( 'NONE', #102677, #25115 ) ;
#41853=FACE_BOUND ( 'NONE', #73738, .T. ) ;
#41854=AXIS2_PLACEMENT_3D ( 'NONE', #2396, #82281, #10920 ) ;
#41856=DIRECTION ( 'NONE',  ( -0.000000000000000000, -1.000000000000000000, -0.000000000000000000 ) ) ;
#41857=DIRECTION ( 'NONE',  ( -0.000000000000000000, 1.000000000000000000, -0.000000000000000000 ) ) ;
#41858=VECTOR ( 'NONE', #89781, 1000.000000000000000 ) ;
#41859=AXIS2_PLACEMENT_3D ( 'NONE', #76615, #17001, #16372 ) ;
#41860=DIRECTION ( 'NONE',  ( -0.000000000000000000, 1.000000000000000000, -0.000000000000000000 ) ) ;
#41861=DIRECTION ( 'NONE',  ( 0.000000000000000000, 0.000000000000000000, -1.000000000000000000 ) ) ;
#41862=CARTESIAN_POINT ( 'NONE',  ( -10.85000000000000142, 12.50000000000000000, -2.165063509461097713 ) ) ;
#41863=ORIENTED_EDGE ( 'NONE', *, *, #108968, .F. ) ;
#41864=CIRCLE ( 'NONE', #125467, 0.1000000000000000472 ) ;
#41865=DIRECTION ( 'NONE',  ( 0.000000000000000000, 0.000000000000000000, -1.000000000000000000 ) ) ;
#41866=EDGE_CURVE ( 'NONE', #119726, #10174, #124138, .T. ) ;
#41867=DIRECTION ( 'NONE',  ( -0.000000000000000000, 1.000000000000000000, -0.000000000000000000 ) ) ;
#41868=AXIS2_PLACEMENT_3D ( 'NONE', #105445, #95621, #125699 ) ;
#41869=VERTEX_POINT ( 'NONE', #38817 ) ;
#41870=ORIENTED_EDGE ( 'NONE', *, *, #95301, .F. ) ;
#41871=FACE_OUTER_BOUND ( 'NONE', #57297, .T. ) ;
#41872=EDGE_CURVE ( 'NONE', #81006, #30789, #67701, .T. ) ;
#41873=LINE ( 'NONE', #92233, #65370 ) ;
#41874=FACE_BOUND ( 'NONE', #42761, .T. ) ;
#41875=EDGE_CURVE ( 'NONE', #35997, #120269, #34281, .T. ) ;
#41876=CARTESIAN_POINT ( 'NONE',  ( 4.199999999999941558, 12.50000000000000000, -4.265033745738164406 ) ) ;
#41877=EDGE_CURVE ( 'NONE', #42325, #62716, #92761, .T. ) ;
#41878=EDGE_CURVE ( 'NONE', #106136, #112609, #79989, .T. ) ;
#41879=ORIENTED_EDGE ( 'NONE', *, *, #78096, .F. ) ;
#41880=DIRECTION ( 'NONE',  ( -4.274815082592931898E-19, -0.9999939076577903929, -0.003490651415223739937 ) ) ;
#41881=EDGE_CURVE ( 'NONE', #17735, #117196, #30076, .T. ) ;
#41882=ADVANCED_FACE ( 'NONE', ( #37506 ), #71931, .T. ) ;
#41884=EDGE_CURVE ( 'NONE', #123363, #20166, #47319, .T. ) ;
#41885=ORIENTED_EDGE ( 'NONE', *, *, #47624, .T. ) ;
#41886=DIRECTION ( 'NONE',  ( 0.000000000000000000, -0.000000000000000000, 1.000000000000000000 ) ) ;
#41887=FACE_OUTER_BOUND ( 'NONE', #4616, .T. ) ;
#41888=CIRCLE ( 'NONE', #10552, 0.06509327318403741736 ) ;
#41889=ORIENTED_EDGE ( 'NONE', *, *, #7306, .F. ) ;
#41890=CARTESIAN_POINT ( 'NONE',  ( 1.649999999999951505, 12.50000000000000000, 2.792790559304612064 ) ) ;
#41891=AXIS2_PLACEMENT_3D ( 'NONE', #124830, #35174, #75708 ) ;
#41892=DIRECTION ( 'NONE',  ( 0.000000000000000000, 0.000000000000000000, -1.000000000000000000 ) ) ;
#41893=EDGE_CURVE ( 'NONE', #12959, #65883, #32227, .T. ) ;
#41894=ORIENTED_EDGE ( 'NONE', *, *, #77977, .F. ) ;
#41895=DIRECTION ( 'NONE',  ( 0.000000000000000000, 0.000000000000000000, 1.000000000000000000 ) ) ;
#41896=AXIS2_PLACEMENT_3D ( 'NONE', #99773, #49398, #129257 ) ;
#41897=AXIS2_PLACEMENT_3D ( 'NONE', #9496, #100449, #19295 ) ;
#41898=DIRECTION ( 'NONE',  ( 0.000000000000000000, 0.000000000000000000, 1.000000000000000000 ) ) ;
#41899=CYLINDRICAL_SURFACE ( 'NONE', #101589, 10.00000000000000000 ) ;
#41900=ORIENTED_EDGE ( 'NONE', *, *, #29087, .F. ) ;
#41901=VERTEX_POINT ( 'NONE', #17845 ) ;
#41902=CARTESIAN_POINT ( 'NONE',  ( -11.64999999999999680, 2.500000000000000000, 7.288010851410849256 ) ) ;
#41903=VERTEX_POINT ( 'NONE', #9317 ) ;
#41904=CARTESIAN_POINT ( 'NONE',  ( -4.600000000000024514, 2.500000000000000000, 3.637306695894644726 ) ) ;
#41905=CARTESIAN_POINT ( 'NONE',  ( 10.64999999999990976, 2.500000000000000000, 1.818653347947321475 ) ) ;
#41906=CARTESIAN_POINT ( 'NONE',  ( 6.849999999999929479, 2.500000000000000000, -2.511473670974877948 ) ) ;
#41907=ORIENTED_EDGE ( 'NONE', *, *, #26180, .T. ) ;
#41908=DIRECTION ( 'NONE',  ( 0.000000000000000000, 0.000000000000000000, 1.000000000000000000 ) ) ;
#41909=CARTESIAN_POINT ( 'NONE',  ( -6.050000000000018474, 2.500000000000000000, 2.511473670974873507 ) ) ;
#41911=CARTESIAN_POINT ( 'NONE',  ( 3.349999999999944578, 2.500000000000000000, -5.902370205355750521 ) ) ;
#41912=DIRECTION ( 'NONE',  ( 0.000000000000000000, -0.000000000000000000, 1.000000000000000000 ) ) ;
#41913=FACE_OUTER_BOUND ( 'NONE', #96057, .T. ) ;
#41914=EDGE_LOOP ( 'NONE', ( #78806, #47984 ) ) ;
#41916=CARTESIAN_POINT ( 'NONE',  ( 15.39999999999989200, 2.500000000000000000, -0.7928203230275543412 ) ) ;
#41917=ORIENTED_EDGE ( 'NONE', *, *, #12546, .T. ) ;
#41919=ORIENTED_EDGE ( 'NONE', *, *, #53114, .T. ) ;
#41920=ORIENTED_EDGE ( 'NONE', *, *, #110180, .F. ) ;
#41921=VERTEX_POINT ( 'NONE', #69516 ) ;
#41922=EDGE_CURVE ( 'NONE', #5094, #47068, #68875, .T. ) ;
#41923=DIRECTION ( 'NONE',  ( 0.000000000000000000, 0.000000000000000000, 1.000000000000000000 ) ) ;
#41924=EDGE_CURVE ( 'NONE', #47526, #78573, #7051, .T. ) ;
#41925=DIRECTION ( 'NONE',  ( -0.000000000000000000, 1.000000000000000000, -0.000000000000000000 ) ) ;
#41926=AXIS2_PLACEMENT_3D ( 'NONE', #121598, #31956, #39856 ) ;
#41927=DIRECTION ( 'NONE',  ( 0.000000000000000000, 0.000000000000000000, -1.000000000000000000 ) ) ;
#41928=EDGE_CURVE ( 'NONE', #123848, #101406, #96948, .T. ) ;
#41930=DIRECTION ( 'NONE',  ( 0.000000000000000000, 1.000000000000000000, 0.000000000000000000 ) ) ;
#41931=DIRECTION ( 'NONE',  ( 0.000000000000000000, -0.000000000000000000, 1.000000000000000000 ) ) ;
#41933=DIRECTION ( 'NONE',  ( -0.000000000000000000, -1.000000000000000000, -0.000000000000000000 ) ) ;
#41934=CARTESIAN_POINT ( 'NONE',  ( 10.44999999999991047, 2.500000000000000000, 2.165063509461097713 ) ) ;
#41935=EDGE_CURVE ( 'NONE', #112874, #115594, #38137, .T. ) ;
#41936=CARTESIAN_POINT ( 'NONE',  ( 5.449999999999936229, 12.50000000000000000, 6.430097255199259010 ) ) ;
#41937=ADVANCED_FACE ( 'NONE', ( #68232 ), #108155, .T. ) ;
#41938=EDGE_CURVE ( 'NONE', #10213, #117937, #23804, .T. ) ;
#41939=VERTEX_POINT ( 'NONE', #48606 ) ;
#41940=EDGE_CURVE ( 'NONE', #23223, #72558, #802, .T. ) ;
#41941=DIRECTION ( 'NONE',  ( -0.000000000000000000, -1.000000000000000000, -0.000000000000000000 ) ) ;
#41942=EDGE_LOOP ( 'NONE', ( #64877, #123521, #52859, #53405 ) ) ;
#41943=EDGE_LOOP ( 'NONE', ( #84388, #14715, #5326, #83135 ) ) ;
#41944=FACE_OUTER_BOUND ( 'NONE', #87620, .T. ) ;
#41945=DIRECTION ( 'NONE',  ( 0.000000000000000000, -0.9999939076577903929, 0.003490651415223739937 ) ) ;
#41946=LINE ( 'NONE', #20996, #36079 ) ;
#41947=EDGE_CURVE ( 'NONE', #27524, #128176, #11369, .T. ) ;
#41948=AXIS2_PLACEMENT_3D ( 'NONE', #2037, #33459, #53724 ) ;
#41949=DIRECTION ( 'NONE',  ( 0.000000000000000000, 0.000000000000000000, -1.000000000000000000 ) ) ;
#41950=CIRCLE ( 'NONE', #106675, 0.09999999999999982514 ) ;
#41951=CARTESIAN_POINT ( 'NONE',  ( -9.400000000000007461, 2.500000000000000000, -0.3464101615137783474 ) ) ;
#41952=DIRECTION ( 'NONE',  ( 0.000000000000000000, 0.000000000000000000, 1.000000000000000000 ) ) ;
#41953=LINE ( 'NONE', #120502, #59281 ) ;
#41954=ORIENTED_EDGE ( 'NONE', *, *, #65848, .T. ) ;
#41955=ORIENTED_EDGE ( 'NONE', *, *, #86029, .T. ) ;
#41956=EDGE_LOOP ( 'NONE', ( #16442, #85205 ) ) ;
#41957=ORIENTED_EDGE ( 'NONE', *, *, #51336, .F. ) ;
#41958=EDGE_CURVE ( 'NONE', #39483, #108866, #113780, .T. ) ;
#41959=VERTEX_POINT ( 'NONE', #72754 ) ;
#41961=CARTESIAN_POINT ( 'NONE',  ( -11.64999999999999680, 2.500000000000000000, 1.472243186433545459 ) ) ;
#41962=DIRECTION ( 'NONE',  ( 0.000000000000000000, 1.000000000000000000, 0.000000000000000000 ) ) ;
#41963=CARTESIAN_POINT ( 'NONE',  ( -3.950000000000024603, 2.500000000000000000, -2.511473670974877948 ) ) ;
#41964=FACE_OUTER_BOUND ( 'NONE', #80078, .T. ) ;
#41965=ORIENTED_EDGE ( 'NONE', *, *, #96694, .F. ) ;
#41966=DIRECTION ( 'NONE',  ( 0.000000000000000000, 1.000000000000000000, 0.000000000000000000 ) ) ;
#41967=DIRECTION ( 'NONE',  ( 0.000000000000000000, 0.000000000000000000, 1.000000000000000000 ) ) ;
#41968=LINE ( 'NONE', #63539, #54127 ) ;
#41969=DIRECTION ( 'NONE',  ( -4.274815082592931898E-19, -0.9999939076577903929, -0.003490651415223739937 ) ) ;
#41970=CARTESIAN_POINT ( 'NONE',  ( -8.750000000000010658, 2.500000000000000000, 2.757883832488649656 ) ) ;
#41971=EDGE_LOOP ( 'NONE', ( #81433, #65441 ) ) ;
#41972=EDGE_CURVE ( 'NONE', #37042, #72947, #76119, .T. ) ;
#41973=ORIENTED_EDGE ( 'NONE', *, *, #68995, .T. ) ;
#41974=ORIENTED_EDGE ( 'NONE', *, *, #27261, .F. ) ;
#41975=VECTOR ( 'NONE', #59671, 1000.000000000000000 ) ;
#41976=DIRECTION ( 'NONE',  ( 0.000000000000000000, 1.000000000000000000, 0.000000000000000000 ) ) ;
#41977=AXIS2_PLACEMENT_3D ( 'NONE', #53362, #2299, #362 ) ;
#41978=VERTEX_POINT ( 'NONE', #50522 ) ;
#41979=CARTESIAN_POINT ( 'NONE',  ( 11.64999999999990266, 2.500000000000000000, -6.495190528383302464 ) ) ;
#41980=CARTESIAN_POINT ( 'NONE',  ( -7.900000000000014566, 12.50000000000000000, -3.637306695894650055 ) ) ;
#41981=AXIS2_PLACEMENT_3D ( 'NONE', #117948, #27626, #67551 ) ;
#41982=CIRCLE ( 'NONE', #2249, 0.06509327318403745899 ) ;
#41983=ORIENTED_EDGE ( 'NONE', *, *, #23518, .T. ) ;
#41985=LINE ( 'NONE', #51811, #120565 ) ;
#41986=ADVANCED_FACE ( 'NONE', ( #10584 ), #99207, .T. ) ;
#41987=DIRECTION ( 'NONE',  ( 0.000000000000000000, 0.000000000000000000, 1.000000000000000000 ) ) ;
#41988=DIRECTION ( 'NONE',  ( 0.000000000000000000, -0.000000000000000000, 1.000000000000000000 ) ) ;
#41989=CARTESIAN_POINT ( 'NONE',  ( -0.6000000000000388356, 12.50000000000000000, 3.983716857408420964 ) ) ;
#41990=ORIENTED_EDGE ( 'NONE', *, *, #36103, .T. ) ;
#41991=EDGE_LOOP ( 'NONE', ( #89938, #1568, #121852, #26616 ) ) ;
#41992=DIRECTION ( 'NONE',  ( -0.000000000000000000, -1.000000000000000000, -0.000000000000000000 ) ) ;
#41993=LINE ( 'NONE', #51822, #64413 ) ;
#41994=CARTESIAN_POINT ( 'NONE',  ( 0.8499999999999557909, 2.500000000000000000, -6.495190528383302464 ) ) ;
#41995=LINE ( 'NONE', #21051, #77302 ) ;
#41998=DIRECTION ( 'NONE',  ( -0.000000000000000000, -1.000000000000000000, -0.000000000000000000 ) ) ;
#41999=CARTESIAN_POINT ( 'NONE',  ( 10.84999999999991260, 12.50000000000000000, 6.560283801567334372 ) ) ;
#42000=DIRECTION ( 'NONE',  ( 0.000000000000000000, 0.000000000000000000, 1.000000000000000000 ) ) ;
#42001=DIRECTION ( 'NONE',  ( 0.000000000000000000, -0.9999939076577903929, 0.003490651415223739937 ) ) ;
#42002=ORIENTED_EDGE ( 'NONE', *, *, #56440, .T. ) ;
#42003=AXIS2_PLACEMENT_3D ( 'NONE', #62097, #89609, #61455 ) ;
#42004=DIRECTION ( 'NONE',  ( -0.000000000000000000, -1.000000000000000000, -0.000000000000000000 ) ) ;
#42005=EDGE_CURVE ( 'NONE', #82577, #93997, #81288, .T. ) ;
#42006=LINE ( 'NONE', #50523, #7648 ) ;
#42007=VERTEX_POINT ( 'NONE', #82586 ) ;
#42008=CARTESIAN_POINT ( 'NONE',  ( 3.949999999999941558, 12.50000000000000000, -1.883746621131363597 ) ) ;
#42009=ORIENTED_EDGE ( 'NONE', *, *, #28739, .F. ) ;
#42010=CONICAL_SURFACE ( 'NONE', #33698, 0.09999999999999982514, 0.003490658503988666988 ) ;
#42011=DIRECTION ( 'NONE',  ( 0.000000000000000000, 1.000000000000000000, 0.000000000000000000 ) ) ;
#42013=VERTEX_POINT ( 'NONE', #90434 ) ;
#42014=DIRECTION ( 'NONE',  ( 0.000000000000000000, 0.000000000000000000, 1.000000000000000000 ) ) ;
#42015=CARTESIAN_POINT ( 'NONE',  ( -12.29999999999999538, 12.50000000000000000, -4.741630453620013341 ) ) ;
#42016=EDGE_CURVE ( 'NONE', #62754, #62269, #103314, .T. ) ;
#42017=ORIENTED_EDGE ( 'NONE', *, *, #10867, .T. ) ;
#42018=EDGE_CURVE ( 'NONE', #16041, #110257, #51193, .T. ) ;
#42019=VERTEX_POINT ( 'NONE', #22382 ) ;
#42020=EDGE_CURVE ( 'NONE', #59954, #63275, #57338, .T. ) ;
#42021=ADVANCED_FACE ( 'NONE', ( #43310 ), #60991, .T. ) ;
#42022=FACE_OUTER_BOUND ( 'NONE', #80407, .T. ) ;
#42023=CARTESIAN_POINT ( 'NONE',  ( -6.250000000000021316, 12.50000000000000000, -1.472243186433550122 ) ) ;
#42024=VECTOR ( 'NONE', #11050, 1000.000000000000000 ) ;
#42025=CARTESIAN_POINT ( 'NONE',  ( -12.94999999999999218, 2.500000000000000000, 2.265063509461101354 ) ) ;
#42027=CIRCLE ( 'NONE', #35768, 0.06509327318403745899 ) ;
#42028=EDGE_CURVE ( 'NONE', #129259, #46131, #49046, .T. ) ;
#42029=DIRECTION ( 'NONE',  ( -0.000000000000000000, -1.000000000000000000, -0.000000000000000000 ) ) ;
#42030=DIRECTION ( 'NONE',  ( -4.274815082592931898E-19, -0.9999939076577903929, -0.003490651415223739937 ) ) ;
#42031=DIRECTION ( 'NONE',  ( 0.000000000000000000, 0.000000000000000000, 1.000000000000000000 ) ) ;
#42032=DIRECTION ( 'NONE',  ( 0.000000000000000000, 1.000000000000000000, 0.000000000000000000 ) ) ;
#42033=DIRECTION ( 'NONE',  ( 0.000000000000000000, 0.000000000000000000, -1.000000000000000000 ) ) ;
#42034=EDGE_CURVE ( 'NONE', #112256, #64883, #115825, .T. ) ;
#42035=CIRCLE ( 'NONE', #19030, 0.09999999999999982514 ) ;
#42036=EDGE_CURVE ( 'NONE', #61413, #50205, #124243, .T. ) ;
#42037=EDGE_CURVE ( 'NONE', #88884, #42322, #113316, .T. ) ;
#42038=ORIENTED_EDGE ( 'NONE', *, *, #19965, .T. ) ;
#42040=DIRECTION ( 'NONE',  ( 0.000000000000000000, 1.000000000000000000, 0.000000000000000000 ) ) ;
#42041=ORIENTED_EDGE ( 'NONE', *, *, #38369, .T. ) ;
#42042=AXIS2_PLACEMENT_3D ( 'NONE', #118163, #120109, #50098 ) ;
#42043=FACE_OUTER_BOUND ( 'NONE', #17564, .T. ) ;
#42044=CARTESIAN_POINT ( 'NONE',  ( 9.599999999999914380, 2.500000000000000000, -4.430127018922202176 ) ) ;
#42045=CARTESIAN_POINT ( 'NONE',  ( 15.59999999999988951, 2.500000000000000000, 0.3464101615137735735 ) ) ;
#42046=ORIENTED_EDGE ( 'NONE', *, *, #102074, .T. ) ;
#42047=VERTEX_POINT ( 'NONE', #92380 ) ;
#42049=FACE_BOUND ( 'NONE', #23711, .T. ) ;
#42050=ORIENTED_EDGE ( 'NONE', *, *, #36315, .F. ) ;
#42051=CARTESIAN_POINT ( 'NONE',  ( -5.400000000000019895, 2.500000000000000000, -2.276824562219559311E-15 ) ) ;
#42052=DIRECTION ( 'NONE',  ( -0.000000000000000000, 1.000000000000000000, -0.000000000000000000 ) ) ;
#42053=LINE ( 'NONE', #91147, #51327 ) ;
#42054=LINE ( 'NONE', #113358, #32687 ) ;
#42055=CARTESIAN_POINT ( 'NONE',  ( 4.549999999999939426, 2.500000000000000000, -6.595190528383302109 ) ) ;
#42056=FACE_OUTER_BOUND ( 'NONE', #70848, .T. ) ;
#42057=DIRECTION ( 'NONE',  ( 0.000000000000000000, 1.000000000000000000, 0.000000000000000000 ) ) ;
#42059=CARTESIAN_POINT ( 'NONE',  ( -12.69999999999999218, 2.500000000000000000, 4.776537180435972196 ) ) ;
#42060=DIRECTION ( 'NONE',  ( -0.000000000000000000, 1.000000000000000000, -0.000000000000000000 ) ) ;
#42061=CARTESIAN_POINT ( 'NONE',  ( -10.45000000000000107, 2.500000000000000000, 2.065063509461097624 ) ) ;
#42062=ORIENTED_EDGE ( 'NONE', *, *, #71744, .F. ) ;
#42063=ORIENTED_EDGE ( 'NONE', *, *, #100635, .F. ) ;
#42064=ORIENTED_EDGE ( 'NONE', *, *, #45093, .F. ) ;
#42065=DIRECTION ( 'NONE',  ( 0.000000000000000000, 0.000000000000000000, -1.000000000000000000 ) ) ;
#42066=ORIENTED_EDGE ( 'NONE', *, *, #20766, .F. ) ;
#42067=DIRECTION ( 'NONE',  ( -0.000000000000000000, -1.000000000000000000, -0.000000000000000000 ) ) ;
#42068=CONICAL_SURFACE ( 'NONE', #16969, 0.1000000000000002554, 0.003490658503988666988 ) ;
#42069=LINE ( 'NONE', #121914, #128028 ) ;
#42070=VECTOR ( 'NONE', #126470, 1000.000000000000000 ) ;
#42071=CIRCLE ( 'NONE', #2329, 0.09999999999999999167 ) ;
#42072=ADVANCED_FACE ( 'NONE', ( #21725 ), #84523, .T. ) ;
#42073=ORIENTED_EDGE ( 'NONE', *, *, #64807, .F. ) ;
#42074=VERTEX_POINT ( 'NONE', #121843 ) ;
#42075=ORIENTED_EDGE ( 'NONE', *, *, #11686, .T. ) ;
#42076=DIRECTION ( 'NONE',  ( -0.000000000000000000, 1.000000000000000000, -0.000000000000000000 ) ) ;
#42077=AXIS2_PLACEMENT_3D ( 'NONE', #36685, #25536, #55010 ) ;
#42078=DIRECTION ( 'NONE',  ( 0.000000000000000000, 0.000000000000000000, -1.000000000000000000 ) ) ;
#42079=AXIS2_PLACEMENT_3D ( 'NONE', #83604, #74423, #93416 ) ;
#42080=CARTESIAN_POINT ( 'NONE',  ( -4.150000000000024336, 2.500000000000000000, 1.472243186433545459 ) ) ;
#42081=CARTESIAN_POINT ( 'NONE',  ( -11.89999999999999680, 2.500000000000000000, -0.3464101615137741841 ) ) ;
#42082=CARTESIAN_POINT ( 'NONE',  ( -4.600000000000028066, 2.500000000000000000, -3.537306695894649966 ) ) ;
#42083=CONICAL_SURFACE ( 'NONE', #6516, 0.1000000000000002554, 0.003490658503988666988 ) ;
#42084=DIRECTION ( 'NONE',  ( 0.000000000000000000, 1.000000000000000000, 0.000000000000000000 ) ) ;
#42085=ORIENTED_EDGE ( 'NONE', *, *, #115060, .T. ) ;
#42086=CARTESIAN_POINT ( 'NONE',  ( -8.550000000000011369, 12.50000000000000000, -2.511473670974877948 ) ) ;
#42087=ORIENTED_EDGE ( 'NONE', *, *, #35843, .T. ) ;
#42088=EDGE_CURVE ( 'NONE', #39107, #86369, #21855, .T. ) ;
#42089=ORIENTED_EDGE ( 'NONE', *, *, #8309, .F. ) ;
#42090=ORIENTED_EDGE ( 'NONE', *, *, #45298, .T. ) ;
#42091=ADVANCED_FACE ( 'NONE', ( #62929 ), #59423, .T. ) ;
#42092=CARTESIAN_POINT ( 'NONE',  ( 8.349999999999923261, 2.500000000000000000, 1.472243186433545459 ) ) ;
#42093=ORIENTED_EDGE ( 'NONE', *, *, #5947, .T. ) ;
#42094=ORIENTED_EDGE ( 'NONE', *, *, #113262, .F. ) ;
#42095=ORIENTED_EDGE ( 'NONE', *, *, #101557, .F. ) ;
#42096=ADVANCED_FACE ( 'NONE', ( #83226 ), #33489, .T. ) ;
#42097=FACE_OUTER_BOUND ( 'NONE', #56079, .T. ) ;
#42098=DIRECTION ( 'NONE',  ( 0.000000000000000000, -0.000000000000000000, 1.000000000000000000 ) ) ;
#42099=PLANE ( 'NONE',  #27553 ) ;
#42100=CARTESIAN_POINT ( 'NONE',  ( 9.399999999999915090, 12.50000000000000000, 4.048810130592458201 ) ) ;
#42101=CARTESIAN_POINT ( 'NONE',  ( 1.049999999999952083, 2.500000000000000000, 6.941600689897073018 ) ) ;
#42102=DIRECTION ( 'NONE',  ( -0.000000000000000000, 1.000000000000000000, -0.000000000000000000 ) ) ;
#42103=AXIS2_PLACEMENT_3D ( 'NONE', #90894, #71918, #49703 ) ;
#42104=VECTOR ( 'NONE', #42775, 1000.000000000000000 ) ;
#42105=EDGE_LOOP ( 'NONE', ( #118833, #87313 ) ) ;
#42106=CARTESIAN_POINT ( 'NONE',  ( -3.150000000000032330, 2.500000000000000000, -6.148780366869526226 ) ) ;
#42107=ORIENTED_EDGE ( 'NONE', *, *, #94180, .T. ) ;
#42108=LINE ( 'NONE', #889, #77549 ) ;
#42110=FACE_OUTER_BOUND ( 'NONE', #101418, .T. ) ;
#42111=VERTEX_POINT ( 'NONE', #125696 ) ;
#42112=AXIS2_PLACEMENT_3D ( 'NONE', #49733, #59569, #89642 ) ;
#42113=CARTESIAN_POINT ( 'NONE',  ( 6.449999999999930012, 2.500000000000000000, 6.841600689897072485 ) ) ;
#42115=CARTESIAN_POINT ( 'NONE',  ( -3.749999999999991118, 2.500000000000000000, -2.065063509461102065 ) ) ;
#42116=EDGE_LOOP ( 'NONE', ( #38336, #78895, #70256, #99610 ) ) ;
#42117=ORIENTED_EDGE ( 'NONE', *, *, #111522, .F. ) ;
#42118=DIRECTION ( 'NONE',  ( 0.000000000000000000, 0.000000000000000000, 1.000000000000000000 ) ) ;
#42119=CARTESIAN_POINT ( 'NONE',  ( -2.300000000000033573, 2.500000000000000000, 4.676537180435972552 ) ) ;
#42120=DIRECTION ( 'NONE',  ( 0.000000000000000000, 0.000000000000000000, 1.000000000000000000 ) ) ;
#42121=DIRECTION ( 'NONE',  ( 0.000000000000000000, 1.000000000000000000, 0.000000000000000000 ) ) ;
#42122=AXIS2_PLACEMENT_3D ( 'NONE', #107691, #106391, #67081 ) ;
#42123=CARTESIAN_POINT ( 'NONE',  ( 6.049999999999930544, 2.500000000000000000, 2.511473670974873507 ) ) ;
#42124=VERTEX_POINT ( 'NONE', #75966 ) ;
#42125=EDGE_CURVE ( 'NONE', #69422, #7039, #85139, .T. ) ;
#42126=DIRECTION ( 'NONE',  ( 0.000000000000000000, 1.000000000000000000, 0.000000000000000000 ) ) ;
#42127=CONICAL_SURFACE ( 'NONE', #21279, 0.09999999999999982514, 0.003490658503988666988 ) ;
#42128=CONICAL_SURFACE ( 'NONE', #115241, 0.09999999999999982514, 0.003490658503988666988 ) ;
#42129=ORIENTED_EDGE ( 'NONE', *, *, #57775, .T. ) ;
#42130=CARTESIAN_POINT ( 'NONE',  ( -7.500000000000016875, 2.500000000000000000, -3.637306695894650055 ) ) ;
#42131=DIRECTION ( 'NONE',  ( -0.000000000000000000, -1.000000000000000000, -0.000000000000000000 ) ) ;
#42132=VECTOR ( 'NONE', #51859, 1000.000000000000000 ) ;
#42133=CONICAL_SURFACE ( 'NONE', #115247, 0.1000000000000002554, 0.003490658503988666988 ) ;
#42134=ADVANCED_FACE ( 'NONE', ( #115216 ), #113966, .T. ) ;
#42135=DIRECTION ( 'NONE',  ( -0.000000000000000000, -1.000000000000000000, -0.000000000000000000 ) ) ;
#42136=CARTESIAN_POINT ( 'NONE',  ( 2.699999999999947331, 12.50000000000000000, -0.3464101615137783474 ) ) ;
#42137=CARTESIAN_POINT ( 'NONE',  ( 14.99999999999992895, 2.500000000000000000, -0.1000000000000022815 ) ) ;
#42138=EDGE_CURVE ( 'NONE', #84736, #4055, #34126, .T. ) ;
#42139=DIRECTION ( 'NONE',  ( 0.000000000000000000, 0.000000000000000000, 1.000000000000000000 ) ) ;
#42140=DIRECTION ( 'NONE',  ( 0.000000000000000000, 0.000000000000000000, -1.000000000000000000 ) ) ;
#42141=VERTEX_POINT ( 'NONE', #93680 ) ;
#42142=CARTESIAN_POINT ( 'NONE',  ( 1.249999999999952038, 2.500000000000000000, -1.472243186433550122 ) ) ;
#42143=DIRECTION ( 'NONE',  ( 0.000000000000000000, 0.000000000000000000, 1.000000000000000000 ) ) ;
#42144=PLANE ( 'NONE',  #49658 ) ;
#42145=ORIENTED_EDGE ( 'NONE', *, *, #92465, .T. ) ;
#42146=EDGE_CURVE ( 'NONE', #64315, #50389, #32330, .T. ) ;
#42147=ORIENTED_EDGE ( 'NONE', *, *, #55823, .T. ) ;
#42148=FACE_OUTER_BOUND ( 'NONE', #15340, .T. ) ;
#42149=ORIENTED_EDGE ( 'NONE', *, *, #25008, .T. ) ;
#42150=EDGE_LOOP ( 'NONE', ( #58384, #8612, #107871, #582 ) ) ;
#42151=DIRECTION ( 'NONE',  ( -0.000000000000000000, -1.000000000000000000, -0.000000000000000000 ) ) ;
#42152=CIRCLE ( 'NONE', #29621, 0.1000000000000000472 ) ;
#42153=CONICAL_SURFACE ( 'NONE', #106975, 0.1000000000000000056, 0.003490658503988666988 ) ;
#42154=CONICAL_SURFACE ( 'NONE', #63078, 0.09999999999999982514, 0.003490658503988666988 ) ;
#42155=EDGE_LOOP ( 'NONE', ( #62028, #14361, #44143, #32727 ) ) ;
#42156=CARTESIAN_POINT ( 'NONE',  ( 1.049999999999952971, 12.50000000000000000, 6.213873640053559022 ) ) ;
#42157=CARTESIAN_POINT ( 'NONE',  ( -8.150000000000012790, 2.500000000000000000, -2.611473670974877592 ) ) ;
#42158=CARTESIAN_POINT ( 'NONE',  ( 18.27284318114731931, 0.4998542452748436227, 4.791717918552973465 ) ) ;
#42159=ORIENTED_EDGE ( 'NONE', *, *, #63493, .F. ) ;
#42160=AXIS2_PLACEMENT_3D ( 'NONE', #39282, #119098, #81118 ) ;
#42161=DIRECTION ( 'NONE',  ( 0.000000000000000000, 0.000000000000000000, 1.000000000000000000 ) ) ;
#42162=EDGE_CURVE ( 'NONE', #38593, #120493, #126367, .T. ) ;
#42163=DIRECTION ( 'NONE',  ( 0.000000000000000000, 0.000000000000000000, 1.000000000000000000 ) ) ;
#42164=AXIS2_PLACEMENT_3D ( 'NONE', #94680, #35772, #123493 ) ;
#42165=VERTEX_POINT ( 'NONE', #55685 ) ;
#42166=CIRCLE ( 'NONE', #115293, 0.06509327318403745899 ) ;
#42167=EDGE_CURVE ( 'NONE', #47326, #114265, #95616, .T. ) ;
#42168=ORIENTED_EDGE ( 'NONE', *, *, #40736, .T. ) ;
#42169=ORIENTED_EDGE ( 'NONE', *, *, #109961, .F. ) ;
#42170=DIRECTION ( 'NONE',  ( 0.000000000000000000, -0.9999939076577903929, 0.003490651415223739937 ) ) ;
#42171=DIRECTION ( 'NONE',  ( 0.000000000000000000, -0.000000000000000000, 1.000000000000000000 ) ) ;
#42172=DIRECTION ( 'NONE',  ( 0.000000000000000000, -0.000000000000000000, 1.000000000000000000 ) ) ;
#42173=EDGE_CURVE ( 'NONE', #17483, #60337, #111718, .T. ) ;
#42174=EDGE_CURVE ( 'NONE', #50142, #51049, #109578, .T. ) ;
#42175=FACE_BOUND ( 'NONE', #76795, .T. ) ;
#42176=ORIENTED_EDGE ( 'NONE', *, *, #75127, .T. ) ;
#42177=EDGE_CURVE ( 'NONE', #85507, #4707, #55287, .T. ) ;
#42178=EDGE_CURVE ( 'NONE', #39225, #70505, #126300, .T. ) ;
#42179=CARTESIAN_POINT ( 'NONE',  ( -2.700000000000029932, 2.500000000000000000, -4.776537180435977525 ) ) ;
#42180=CARTESIAN_POINT ( 'NONE',  ( 1.449999999999951328, 2.500000000000000000, -1.818653347947326138 ) ) ;
#42181=ORIENTED_EDGE ( 'NONE', *, *, #73994, .F. ) ;
#42182=LINE ( 'NONE', #64389, #122046 ) ;
#42183=CARTESIAN_POINT ( 'NONE',  ( 1.899999999999951283, 2.500000000000000000, -0.3464101615137782364 ) ) ;
#42184=EDGE_CURVE ( 'NONE', #2990, #102929, #117964, .T. ) ;
#42185=DIRECTION ( 'NONE',  ( 0.000000000000000000, 0.000000000000000000, 1.000000000000000000 ) ) ;
#42186=DIRECTION ( 'NONE',  ( 0.000000000000000000, 0.000000000000000000, 1.000000000000000000 ) ) ;
#42187=DIRECTION ( 'NONE',  ( -0.000000000000000000, 1.000000000000000000, -0.000000000000000000 ) ) ;
#42188=ADVANCED_FACE ( 'NONE', ( #4624 ), #13411, .T. ) ;
#42189=DIRECTION ( 'NONE',  ( 0.000000000000000000, 1.000000000000000000, 0.000000000000000000 ) ) ;
#42190=FACE_OUTER_BOUND ( 'NONE', #123540, .T. ) ;
#42191=AXIS2_PLACEMENT_3D ( 'NONE', #37144, #28610, #56739 ) ;
#42192=CIRCLE ( 'NONE', #115314, 0.09999999999999982514 ) ;
#42193=EDGE_CURVE ( 'NONE', #75709, #4289, #72021, .T. ) ;
#42195=ORIENTED_EDGE ( 'NONE', *, *, #46304, .T. ) ;
#42196=ORIENTED_EDGE ( 'NONE', *, *, #104762, .F. ) ;
#42197=EDGE_LOOP ( 'NONE', ( #96529, #45458 ) ) ;
#42198=ORIENTED_EDGE ( 'NONE', *, *, #121474, .T. ) ;
#42199=DIRECTION ( 'NONE',  ( -0.000000000000000000, 1.000000000000000000, -0.000000000000000000 ) ) ;
#42200=FACE_OUTER_BOUND ( 'NONE', #110832, .T. ) ;
#42201=CARTESIAN_POINT ( 'NONE',  ( -1.050000000000037792, 2.500000000000000000, 6.148780366869520009 ) ) ;
#42202=VERTEX_POINT ( 'NONE', #55042 ) ;
#42203=FACE_BOUND ( 'NONE', #5951, .T. ) ;
#42204=EDGE_CURVE ( 'NONE', #74055, #6638, #86572, .T. ) ;
#42205=CARTESIAN_POINT ( 'NONE',  ( -4.999999999999990230, 2.500000000000000000, -4.330127018922201643 ) ) ;
#42206=DIRECTION ( 'NONE',  ( -0.000000000000000000, -1.000000000000000000, -0.000000000000000000 ) ) ;
#42207=CIRCLE ( 'NONE', #107015, 0.1000000000000002554 ) ;
#42208=AXIS2_PLACEMENT_3D ( 'NONE', #83335, #103615, #64320 ) ;
#42209=CARTESIAN_POINT ( 'NONE',  ( -2.700000000000030820, 12.50000000000000000, -3.983716857408426293 ) ) ;
#42210=VECTOR ( 'NONE', #58068, 1000.000000000000000 ) ;
#42211=AXIS2_PLACEMENT_3D ( 'NONE', #45284, #15140, #45932 ) ;
#42212=CARTESIAN_POINT ( 'NONE',  ( -1.850000000000033396, 2.500000000000000000, -1.918653347947325782 ) ) ;
#42213=DIRECTION ( 'NONE',  ( 0.000000000000000000, 1.000000000000000000, 0.000000000000000000 ) ) ;
#42215=CARTESIAN_POINT ( 'NONE',  ( -8.100000000000013856, 12.50000000000000000, -0.3464101615137782364 ) ) ;
#42216=DIRECTION ( 'NONE',  ( 0.000000000000000000, 1.000000000000000000, 0.000000000000000000 ) ) ;
#42217=PLANE ( 'NONE',  #14117 ) ;
#42218=VECTOR ( 'NONE', #56613, 1000.000000000000000 ) ;
#42219=EDGE_LOOP ( 'NONE', ( #89363, #76426 ) ) ;
#42220=DIRECTION ( 'NONE',  ( -4.274815082592931898E-19, -0.9999939076577903929, -0.003490651415223739937 ) ) ;
#42221=ORIENTED_EDGE ( 'NONE', *, *, #45900, .T. ) ;
#42222=ORIENTED_EDGE ( 'NONE', *, *, #18809, .T. ) ;
#42223=ORIENTED_EDGE ( 'NONE', *, *, #97147, .F. ) ;
#42224=AXIS2_PLACEMENT_3D ( 'NONE', #100303, #79378, #38156 ) ;
#42225=EDGE_LOOP ( 'NONE', ( #57535, #111335 ) ) ;
#42226=AXIS2_PLACEMENT_3D ( 'NONE', #14535, #25655, #64927 ) ;
#42227=AXIS2_PLACEMENT_3D ( 'NONE', #57997, #118835, #78290 ) ;
#42230=ORIENTED_EDGE ( 'NONE', *, *, #104756, .F. ) ;
#42231=VERTEX_POINT ( 'NONE', #124433 ) ;
#42232=AXIS2_PLACEMENT_3D ( 'NONE', #68398, #108325, #8823 ) ;
#42233=DIRECTION ( 'NONE',  ( 0.000000000000000000, -0.9999939076577903929, 0.003490651415223739937 ) ) ;
#42234=CIRCLE ( 'NONE', #123767, 0.1000000000000002554 ) ;
#42235=CARTESIAN_POINT ( 'NONE',  ( 12.49999999999993960, 12.50000000000000000, -4.395220292106239768 ) ) ;
#42236=CARTESIAN_POINT ( 'NONE',  ( 11.44999999999990870, 2.500000000000000000, 6.741600689897071952 ) ) ;
#42237=CARTESIAN_POINT ( 'NONE',  ( 12.49999999999990052, 2.500000000000000000, 0.7928203230275495672 ) ) ;
#42238=ORIENTED_EDGE ( 'NONE', *, *, #124578, .T. ) ;
#42239=DIRECTION ( 'NONE',  ( -0.000000000000000000, 1.000000000000000000, -0.000000000000000000 ) ) ;
#42240=ORIENTED_EDGE ( 'NONE', *, *, #65784, .F. ) ;
#42241=EDGE_CURVE ( 'NONE', #88360, #109444, #34779, .T. ) ;
#42243=DIRECTION ( 'NONE',  ( 0.000000000000000000, 1.000000000000000000, 0.000000000000000000 ) ) ;
#42244=EDGE_CURVE ( 'NONE', #72184, #116662, #65737, .T. ) ;
#42245=FACE_OUTER_BOUND ( 'NONE', #13200, .T. ) ;
#42246=ORIENTED_EDGE ( 'NONE', *, *, #51244, .F. ) ;
#42247=EDGE_LOOP ( 'NONE', ( #15995, #104085, #91691, #89047 ) ) ;
#42248=FACE_OUTER_BOUND ( 'NONE', #65052, .T. ) ;
#42249=CARTESIAN_POINT ( 'NONE',  ( -0.8500000000000390576, 2.500000000000000000, -2.165063509461101710 ) ) ;
#42250=FACE_OUTER_BOUND ( 'NONE', #84658, .T. ) ;
#42251=CONICAL_SURFACE ( 'NONE', #40196, 0.1000000000000002554, 0.003490658503988666988 ) ;
#42252=DIRECTION ( 'NONE',  ( 0.000000000000000000, -0.000000000000000000, 1.000000000000000000 ) ) ;
#42253=CIRCLE ( 'NONE', #12972, 0.09999999999999982514 ) ;
#42254=AXIS2_PLACEMENT_3D ( 'NONE', #57721, #28251, #26328 ) ;
#42255=CARTESIAN_POINT ( 'NONE',  ( -0.6000000000000383915, 12.50000000000000000, -4.676537180435977881 ) ) ;
#42256=ORIENTED_EDGE ( 'NONE', *, *, #101862, .T. ) ;
#42257=CARTESIAN_POINT ( 'NONE',  ( 2.099999999999949463, 2.500000000000000000, 0.7928203230275495672 ) ) ;
#42258=CIRCLE ( 'NONE', #115373, 0.09999999999999982514 ) ;
#42259=CIRCLE ( 'NONE', #127929, 0.1000000000000002554 ) ;
#42260=ORIENTED_EDGE ( 'NONE', *, *, #107649, .F. ) ;
#42261=CARTESIAN_POINT ( 'NONE',  ( 17.50000000000000000, 2.499999999999999556, -0.3333333333333299286 ) ) ;
#42262=CONICAL_SURFACE ( 'NONE', #115376, 0.09999999999999999167, 0.003490658503988666988 ) ;
#42263=DIRECTION ( 'NONE',  ( -0.000000000000000000, -1.000000000000000000, -0.000000000000000000 ) ) ;
#42264=DIRECTION ( 'NONE',  ( -0.000000000000000000, 1.000000000000000000, -0.000000000000000000 ) ) ;
#42265=CIRCLE ( 'NONE', #115378, 1.000000000000000888 ) ;
#42266=AXIS2_PLACEMENT_3D ( 'NONE', #76112, #95111, #16521 ) ;
#42267=CARTESIAN_POINT ( 'NONE',  ( 11.04999999999990656, 12.50000000000000000, -6.148780366869526226 ) ) ;
#42268=CARTESIAN_POINT ( 'NONE',  ( -4.076600168545496672E-14, 2.500000000000000000, -5.022947341949754119 ) ) ;
#42269=ORIENTED_EDGE ( 'NONE', *, *, #124658, .F. ) ;
#42270=AXIS2_PLACEMENT_3D ( 'NONE', #125491, #105858, #37129 ) ;
#42271=DIRECTION ( 'NONE',  ( -0.000000000000000000, -1.000000000000000000, -0.000000000000000000 ) ) ;
#42272=CARTESIAN_POINT ( 'NONE',  ( 10.84999999999990905, 12.50000000000000000, -6.495190528383302464 ) ) ;
#42273=ORIENTED_EDGE ( 'NONE', *, *, #44030, .F. ) ;
#42274=VERTEX_POINT ( 'NONE', #75320 ) ;
#42276=CARTESIAN_POINT ( 'NONE',  ( -15.39999999999997904, 2.500000000000000000, -0.5928203230275518321 ) ) ;
#42277=PLANE ( 'NONE',  #53368 ) ;
#42278=CARTESIAN_POINT ( 'NONE',  ( 14.14999999999989733, 12.50000000000000000, 1.472243186433545459 ) ) ;
#42279=DIRECTION ( 'NONE',  ( -0.000000000000000000, 1.000000000000000000, -0.000000000000000000 ) ) ;
#42281=DIRECTION ( 'NONE',  ( 0.000000000000000000, 1.000000000000000000, 0.000000000000000000 ) ) ;
#42282=DIRECTION ( 'NONE',  ( 0.000000000000000000, 0.000000000000000000, 1.000000000000000000 ) ) ;
#42283=FACE_OUTER_BOUND ( 'NONE', #100640, .T. ) ;
#42284=AXIS2_PLACEMENT_3D ( 'NONE', #25205, #92027, #72403 ) ;
#42285=DIRECTION ( 'NONE',  ( 0.000000000000000000, -0.9999939076577903929, 0.003490651415223739937 ) ) ;
#42286=EDGE_LOOP ( 'NONE', ( #120249, #111869 ) ) ;
#42287=CARTESIAN_POINT ( 'NONE',  ( -11.44999999999999751, 12.50000000000000000, 2.511473670974873507 ) ) ;
#42288=ADVANCED_FACE ( 'NONE', ( #119124 ), #9167, .T. ) ;
#42289=CARTESIAN_POINT ( 'NONE',  ( 10.39999999999991154, 2.500000000000000000, -3.737306695894649700 ) ) ;
#42291=CARTESIAN_POINT ( 'NONE',  ( -1.250000000000037970, 12.50000000000000000, 2.922977105672686982 ) ) ;
#42292=CARTESIAN_POINT ( 'NONE',  ( -9.999999999999969802, 2.500000000000000000, 4.330127018922196314 ) ) ;
#42293=AXIS2_PLACEMENT_3D ( 'NONE', #86743, #126678, #47473 ) ;
#42294=CONICAL_SURFACE ( 'NONE', #31826, 0.09999999999999982514, 0.003490658503988666988 ) ;
#42295=ORIENTED_EDGE ( 'NONE', *, *, #100137, .T. ) ;
#42296=DIRECTION ( 'NONE',  ( -4.274815082592931898E-19, -0.9999939076577903929, -0.003490651415223739937 ) ) ;
#42297=AXIS2_PLACEMENT_3D ( 'NONE', #98283, #39403, #38087 ) ;
#42298=AXIS2_PLACEMENT_3D ( 'NONE', #52739, #56441, #106824 ) ;
#42299=CARTESIAN_POINT ( 'NONE',  ( -8.350000000000008527, 2.500000000000000000, 7.288010851410849256 ) ) ;
#42300=CARTESIAN_POINT ( 'NONE',  ( -5.850000000000018296, 2.500000000000000000, 1.372243186433545370 ) ) ;
#42301=ORIENTED_EDGE ( 'NONE', *, *, #93303, .F. ) ;
#42302=EDGE_CURVE ( 'NONE', #48001, #90845, #120043, .T. ) ;
#42303=CIRCLE ( 'NONE', #2560, 0.06509327318403745899 ) ;
#42304=ORIENTED_EDGE ( 'NONE', *, *, #2313, .T. ) ;
#42305=DIRECTION ( 'NONE',  ( -4.274815082592931898E-19, -0.9999939076577903929, -0.003490651415223739937 ) ) ;
#42306=AXIS2_PLACEMENT_3D ( 'NONE', #103516, #83860, #104156 ) ;
#42307=ORIENTED_EDGE ( 'NONE', *, *, #96025, .T. ) ;
#42308=CONICAL_SURFACE ( 'NONE', #69480, 0.09999999999999982514, 0.003490658503988666988 ) ;
#42309=VECTOR ( 'NONE', #44498, 1000.000000000000000 ) ;
#42310=ORIENTED_EDGE ( 'NONE', *, *, #39816, .F. ) ;
#42311=CARTESIAN_POINT ( 'NONE',  ( 11.84999999999990372, 12.50000000000000000, -6.148780366869526226 ) ) ;
#42312=AXIS2_PLACEMENT_3D ( 'NONE', #11088, #100754, #39315 ) ;
#42313=CARTESIAN_POINT ( 'NONE',  ( 19.51231976789321720, 0.5900868802296501681, -4.348342248682749656 ) ) ;
#42314=DIRECTION ( 'NONE',  ( 0.000000000000000000, -0.9999939076577903929, 0.003490651415223739937 ) ) ;
#42315=CARTESIAN_POINT ( 'NONE',  ( -3.150000000000030109, 12.50000000000000000, -2.576566944158915184 ) ) ;
#42316=ORIENTED_EDGE ( 'NONE', *, *, #38479, .F. ) ;
#42317=CONICAL_SURFACE ( 'NONE', #90410, 0.1000000000000002554, 0.003490658503988666988 ) ;
#42318=DIRECTION ( 'NONE',  ( 0.000000000000000000, -0.000000000000000000, 1.000000000000000000 ) ) ;
#42319=ORIENTED_EDGE ( 'NONE', *, *, #69634, .T. ) ;
#42322=VERTEX_POINT ( 'NONE', #106707 ) ;
#42323=EDGE_CURVE ( 'NONE', #17427, #51388, #99295, .T. ) ;
#42324=ORIENTED_EDGE ( 'NONE', *, *, #71727, .F. ) ;
#42325=VERTEX_POINT ( 'NONE', #96894 ) ;
#42326=ORIENTED_EDGE ( 'NONE', *, *, #113486, .T. ) ;
#42327=DIRECTION ( 'NONE',  ( 0.000000000000000000, 1.000000000000000000, 0.000000000000000000 ) ) ;
#42328=CARTESIAN_POINT ( 'NONE',  ( 16.31212831497987281, 1.500000000000323297, 6.358242018216644809 ) ) ;
#42329=DIRECTION ( 'NONE',  ( 0.000000000000000000, 0.000000000000000000, -1.000000000000000000 ) ) ;
#42330=EDGE_CURVE ( 'NONE', #53498, #93285, #48444, .T. ) ;
#42331=FACE_BOUND ( 'NONE', #111651, .T. ) ;
#42332=ORIENTED_EDGE ( 'NONE', *, *, #83726, .F. ) ;
#42334=ADVANCED_FACE ( 'NONE', ( #88348 ), #47165, .T. ) ;
#42335=DIRECTION ( 'NONE',  ( 0.000000000000000000, 1.000000000000000000, 0.000000000000000000 ) ) ;
#42336=CARTESIAN_POINT ( 'NONE',  ( 3.149999999999944400, 2.500000000000000000, 2.511473670974873507 ) ) ;
#42337=VECTOR ( 'NONE', #109639, 1000.000000000000000 ) ;
#42338=AXIS2_PLACEMENT_3D ( 'NONE', #97432, #36610, #86971 ) ;
#42339=EDGE_CURVE ( 'NONE', #39960, #54236, #79834, .T. ) ;
#42340=CARTESIAN_POINT ( 'NONE',  ( 6.449999999999933564, 2.500000000000000000, -6.941600689897078347 ) ) ;
#42341=AXIS2_PLACEMENT_3D ( 'NONE', #22948, #23578, #42601 ) ;
#42342=EDGE_CURVE ( 'NONE', #54324, #85725, #39308, .T. ) ;
#42343=DIRECTION ( 'NONE',  ( 0.000000000000000000, 0.000000000000000000, 1.000000000000000000 ) ) ;
#42344=ADVANCED_FACE ( 'NONE', ( #58278 ), #68723, .T. ) ;
#42345=DIRECTION ( 'NONE',  ( 0.000000000000000000, 0.000000000000000000, -1.000000000000000000 ) ) ;
#42346=AXIS2_PLACEMENT_3D ( 'NONE', #95549, #16312, #56255 ) ;
#42347=AXIS2_PLACEMENT_3D ( 'NONE', #25361, #77062, #116322 ) ;
#42348=CARTESIAN_POINT ( 'NONE',  ( -1.650000000000035660, 12.50000000000000000, 7.188010851410848723 ) ) ;
#42349=EDGE_CURVE ( 'NONE', #123082, #117024, #59520, .T. ) ;
#42350=ORIENTED_EDGE ( 'NONE', *, *, #80467, .F. ) ;
#42351=ORIENTED_EDGE ( 'NONE', *, *, #91059, .T. ) ;
#42352=ORIENTED_EDGE ( 'NONE', *, *, #8881, .T. ) ;
#42353=VERTEX_POINT ( 'NONE', #108005 ) ;
#42354=ORIENTED_EDGE ( 'NONE', *, *, #73892, .T. ) ;
#42356=CIRCLE ( 'NONE', #117532, 1.000000000000000444 ) ;
#42357=LINE ( 'NONE', #33813, #73785 ) ;
#42358=VERTEX_POINT ( 'NONE', #17008 ) ;
#42359=FACE_BOUND ( 'NONE', #11392, .T. ) ;
#42360=EDGE_CURVE ( 'NONE', #41081, #20554, #42885, .T. ) ;
#42361=AXIS2_PLACEMENT_3D ( 'NONE', #77671, #117576, #27936 ) ;
#42362=CARTESIAN_POINT ( 'NONE',  ( 4.599999999999936584, 12.50000000000000000, 3.637306695894644726 ) ) ;
#42363=ORIENTED_EDGE ( 'NONE', *, *, #28012, .T. ) ;
#42364=CARTESIAN_POINT ( 'NONE',  ( -4.150000000000025224, 2.500000000000000000, 5.702370205355745014 ) ) ;
#42365=DIRECTION ( 'NONE',  ( -4.274815082592931898E-19, -0.9999939076577903929, -0.003490651415223739937 ) ) ;
#42366=CARTESIAN_POINT ( 'NONE',  ( 5.849999999999933920, 2.500000000000000000, 5.902370205355745192 ) ) ;
#42367=EDGE_LOOP ( 'NONE', ( #22922, #22195, #4388, #9250 ) ) ;
#42368=DIRECTION ( 'NONE',  ( 0.000000000000000000, 1.000000000000000000, 0.000000000000000000 ) ) ;
#42369=CONICAL_SURFACE ( 'NONE', #115501, 0.09999999999999999167, 0.003490658503988666988 ) ;
#42370=ORIENTED_EDGE ( 'NONE', *, *, #93610, .T. ) ;
#42371=EDGE_LOOP ( 'NONE', ( #29815, #118430 ) ) ;
#42372=ORIENTED_EDGE ( 'NONE', *, *, #53539, .F. ) ;
#42373=CARTESIAN_POINT ( 'NONE',  ( -3.350000000000028511, 2.500000000000000000, 1.472243186433545459 ) ) ;
#42374=CARTESIAN_POINT ( 'NONE',  ( -7.900000000000014566, 2.500000000000000000, -4.922947341949753586 ) ) ;
#42375=CARTESIAN_POINT ( 'NONE',  ( 13.94999999999989626, 2.500000000000000000, 2.411473670974873862 ) ) ;
#42376=ORIENTED_EDGE ( 'NONE', *, *, #86841, .F. ) ;
#42377=CARTESIAN_POINT ( 'NONE',  ( 3.349999999999941913, 12.50000000000000000, 6.430097255199259010 ) ) ;
#42378=AXIS2_PLACEMENT_3D ( 'NONE', #66428, #51334, #20565 ) ;
#42379=AXIS2_PLACEMENT_3D ( 'NONE', #69710, #7550, #78906 ) ;
#42380=CARTESIAN_POINT ( 'NONE',  ( -4.350000000000027178, 12.50000000000000000, -6.083687093685488989 ) ) ;
#42381=DIRECTION ( 'NONE',  ( 0.000000000000000000, 0.000000000000000000, -1.000000000000000000 ) ) ;
#42382=CARTESIAN_POINT ( 'NONE',  ( 6.849999999999930367, 12.50000000000000000, -6.906693963081115939 ) ) ;
#42384=ORIENTED_EDGE ( 'NONE', *, *, #63595, .F. ) ;
#42385=FACE_OUTER_BOUND ( 'NONE', #49353, .T. ) ;
#42386=CONICAL_SURFACE ( 'NONE', #6743, 0.09999999999999982514, 0.003490658503988666988 ) ;
#42387=EDGE_LOOP ( 'NONE', ( #66407, #98271 ) ) ;
#42388=DIRECTION ( 'NONE',  ( -0.000000000000000000, -1.000000000000000000, -0.000000000000000000 ) ) ;
#42389=CONICAL_SURFACE ( 'NONE', #11059, 0.1000000000000002554, 0.003490658503988666988 ) ;
#42390=AXIS2_PLACEMENT_3D ( 'NONE', #4670, #4046, #113360 ) ;
#42391=ORIENTED_EDGE ( 'NONE', *, *, #86940, .T. ) ;
#42392=AXIS2_PLACEMENT_3D ( 'NONE', #31045, #121323, #81419 ) ;
#42393=EDGE_CURVE ( 'NONE', #88884, #46382, #88817, .T. ) ;
#42394=ORIENTED_EDGE ( 'NONE', *, *, #102696, .T. ) ;
#42395=DIRECTION ( 'NONE',  ( 0.000000000000000000, 1.000000000000000000, 0.000000000000000000 ) ) ;
#42396=FACE_OUTER_BOUND ( 'NONE', #9386, .T. ) ;
#42397=CARTESIAN_POINT ( 'NONE',  ( -14.14999999999998614, 12.50000000000000000, -2.857883832488651521 ) ) ;
#42398=DIRECTION ( 'NONE',  ( -4.274815082592931898E-19, -0.9999939076577903929, -0.003490651415223739937 ) ) ;
#42399=DIRECTION ( 'NONE',  ( -4.274815082592931898E-19, -0.9999939076577903929, -0.003490651415223739937 ) ) ;
#42400=CIRCLE ( 'NONE', #111319, 0.09999999999999982514 ) ;
#42401=ORIENTED_EDGE ( 'NONE', *, *, #5693, .T. ) ;
#42402=EDGE_LOOP ( 'NONE', ( #92130, #19254 ) ) ;
#42403=CIRCLE ( 'NONE', #109285, 0.1000000000000002554 ) ;
#42404=EDGE_CURVE ( 'NONE', #56648, #102123, #46977, .T. ) ;
#42406=DIRECTION ( 'NONE',  ( 0.000000000000000000, -0.9999939076577903929, 0.003490651415223739937 ) ) ;
#42407=CONICAL_SURFACE ( 'NONE', #100974, 0.1000000000000002554, 0.003490658503988666988 ) ;
#42408=CIRCLE ( 'NONE', #23612, 0.06509327318403745899 ) ;
#42409=CIRCLE ( 'NONE', #36146, 0.06509327318403745899 ) ;
#42410=DIRECTION ( 'NONE',  ( 0.000000000000000000, 0.000000000000000000, 1.000000000000000000 ) ) ;
#42411=ORIENTED_EDGE ( 'NONE', *, *, #98927, .T. ) ;
#42412=ORIENTED_EDGE ( 'NONE', *, *, #35053, .T. ) ;
#42413=ORIENTED_EDGE ( 'NONE', *, *, #67624, .F. ) ;
#42414=DIRECTION ( 'NONE',  ( 0.000000000000000000, 0.000000000000000000, 1.000000000000000000 ) ) ;
#42415=AXIS2_PLACEMENT_3D ( 'NONE', #61517, #11749, #82449 ) ;
#42416=ORIENTED_EDGE ( 'NONE', *, *, #72050, .F. ) ;
#42417=FACE_OUTER_BOUND ( 'NONE', #81666, .T. ) ;
#42418=FACE_OUTER_BOUND ( 'NONE', #112007, .T. ) ;
#42419=DIRECTION ( 'NONE',  ( 0.000000000000000000, -0.9999939076577903929, 0.003490651415223739937 ) ) ;
#42420=ORIENTED_EDGE ( 'NONE', *, *, #8631, .F. ) ;
#42421=CONICAL_SURFACE ( 'NONE', #69590, 0.09999999999999982514, 0.003490658503988666988 ) ;
#42422=DIRECTION ( 'NONE',  ( 0.000000000000000000, 1.000000000000000000, 0.000000000000000000 ) ) ;
#42423=LINE ( 'NONE', #101338, #2662 ) ;
#42424=CARTESIAN_POINT ( 'NONE',  ( 7.299999999999926104, 12.50000000000000000, -3.983716857408426293 ) ) ;
#42425=CARTESIAN_POINT ( 'NONE',  ( -0.6000000000000323963, 2.500000000000000000, 0.3464101615137759604 ) ) ;
#42426=DIRECTION ( 'NONE',  ( 0.000000000000000000, 0.000000000000000000, 1.000000000000000000 ) ) ;
#42427=ORIENTED_EDGE ( 'NONE', *, *, #40470, .F. ) ;
#42428=DIRECTION ( 'NONE',  ( -1.000000000000000000, -0.000000000000000000, -0.000000000000000000 ) ) ;
#42429=DIRECTION ( 'NONE',  ( 0.000000000000000000, 0.000000000000000000, 1.000000000000000000 ) ) ;
#42430=EDGE_LOOP ( 'NONE', ( #79271, #63940 ) ) ;
#42431=VERTEX_POINT ( 'NONE', #67408 ) ;
#42432=AXIS2_PLACEMENT_3D ( 'NONE', #108073, #33701, #73612 ) ;
#42433=CONICAL_SURFACE ( 'NONE', #25688, 0.09999999999999982514, 0.003490658503988666988 ) ;
#42435=LINE ( 'NONE', #51611, #69902 ) ;
#42436=DIRECTION ( 'NONE',  ( 0.000000000000000000, 1.000000000000000000, 0.000000000000000000 ) ) ;
#42437=CARTESIAN_POINT ( 'NONE',  ( -6.900000000000015454, 2.500000000000000000, 3.983716857408420076 ) ) ;
#42438=DIRECTION ( 'NONE',  ( 0.000000000000000000, 0.000000000000000000, 1.000000000000000000 ) ) ;
#42439=ADVANCED_FACE ( 'NONE', ( #107363 ), #89024, .T. ) ;
#42440=CIRCLE ( 'NONE', #13449, 0.06509327318403745899 ) ;
#42441=DIRECTION ( 'NONE',  ( 0.000000000000000000, 0.000000000000000000, 1.000000000000000000 ) ) ;
#42442=AXIS2_PLACEMENT_3D ( 'NONE', #62802, #32714, #121069 ) ;
#42443=DIRECTION ( 'NONE',  ( 0.000000000000000000, 0.000000000000000000, -1.000000000000000000 ) ) ;
#42444=CARTESIAN_POINT ( 'NONE',  ( -2.050000000000033129, 2.500000000000000000, 2.065063509461097624 ) ) ;
#42445=CONICAL_SURFACE ( 'NONE', #69612, 0.1000000000000000472, 0.003490658503988666988 ) ;
#42446=AXIS2_PLACEMENT_3D ( 'NONE', #25188, #55943, #76243 ) ;
#42447=ADVANCED_FACE ( 'NONE', ( #109296 ), #61645, .T. ) ;
#42448=CARTESIAN_POINT ( 'NONE',  ( 2.899999999999944844, 12.50000000000000000, 3.637306695894644726 ) ) ;
#42449=EDGE_CURVE ( 'NONE', #95328, #125928, #118062, .T. ) ;
#42450=ORIENTED_EDGE ( 'NONE', *, *, #105442, .F. ) ;
#42451=CIRCLE ( 'NONE', #15216, 0.06509327318403745899 ) ;
#42452=ORIENTED_EDGE ( 'NONE', *, *, #92160, .T. ) ;
#42453=CIRCLE ( 'NONE', #61218, 0.1000000000000002554 ) ;
#42454=AXIS2_PLACEMENT_3D ( 'NONE', #97175, #95249, #35056 ) ;
#42455=ORIENTED_EDGE ( 'NONE', *, *, #12762, .F. ) ;
#42456=CONICAL_SURFACE ( 'NONE', #123999, 0.1000000000000002554, 0.003490658503988666988 ) ;
#42457=ADVANCED_FACE ( 'NONE', ( #60227 ), #116009, .T. ) ;
#42458=VERTEX_POINT ( 'NONE', #61509 ) ;
#42459=ADVANCED_FACE ( 'NONE', ( #94638 ), #90879, .T. ) ;
#42460=DIRECTION ( 'NONE',  ( 0.000000000000000000, 0.000000000000000000, 1.000000000000000000 ) ) ;
#42461=DIRECTION ( 'NONE',  ( 0.000000000000000000, 0.000000000000000000, -1.000000000000000000 ) ) ;
#42462=CONICAL_SURFACE ( 'NONE', #63377, 0.1000000000000002554, 0.003490658503988666988 ) ;
#42463=ORIENTED_EDGE ( 'NONE', *, *, #83554, .T. ) ;
#42464=CARTESIAN_POINT ( 'NONE',  ( 12.49999999999990408, 12.50000000000000000, 4.957854068765711553 ) ) ;
#42465=EDGE_CURVE ( 'NONE', #97094, #37017, #80429, .T. ) ;
#42466=DIRECTION ( 'NONE',  ( 0.000000000000000000, 0.000000000000000000, 1.000000000000000000 ) ) ;
#42467=DIRECTION ( 'NONE',  ( 0.000000000000000000, -0.9999939076577903929, 0.003490651415223739937 ) ) ;
#42468=ORIENTED_EDGE ( 'NONE', *, *, #27082, .T. ) ;
#42469=ADVANCED_FACE ( 'NONE', ( #4967 ), #65825, .T. ) ;
#42470=CARTESIAN_POINT ( 'NONE',  ( -4.150000000000024336, 2.500000000000000000, 1.472243186433545459 ) ) ;
#42471=CARTESIAN_POINT ( 'NONE',  ( -13.74999999999998757, 2.500000000000000000, -2.857883832488651521 ) ) ;
#42472=EDGE_LOOP ( 'NONE', ( #45860, #29040, #107385, #59336 ) ) ;
#42473=ORIENTED_EDGE ( 'NONE', *, *, #18874, .F. ) ;
#42474=ORIENTED_EDGE ( 'NONE', *, *, #10823, .T. ) ;
#42475=ORIENTED_EDGE ( 'NONE', *, *, #32308, .T. ) ;
#42476=DIRECTION ( 'NONE',  ( 0.000000000000000000, 0.000000000000000000, -1.000000000000000000 ) ) ;
#42477=DIRECTION ( 'NONE',  ( 0.000000000000000000, 0.000000000000000000, -1.000000000000000000 ) ) ;
#42478=CONICAL_SURFACE ( 'NONE', #96729, 0.1000000000000002554, 0.003490658503988666988 ) ;
#42479=DIRECTION ( 'NONE',  ( 0.000000000000000000, 0.000000000000000000, 1.000000000000000000 ) ) ;
#42480=AXIS2_PLACEMENT_3D ( 'NONE', #34959, #85949, #65014 ) ;
#42483=VERTEX_POINT ( 'NONE', #11741 ) ;
#42484=DIRECTION ( 'NONE',  ( -0.000000000000000000, -1.000000000000000000, -0.000000000000000000 ) ) ;
#42485=ORIENTED_EDGE ( 'NONE', *, *, #74813, .F. ) ;
#42486=DIRECTION ( 'NONE',  ( 0.000000000000000000, 0.000000000000000000, 1.000000000000000000 ) ) ;
#42487=DIRECTION ( 'NONE',  ( 0.000000000000000000, 1.000000000000000000, 0.000000000000000000 ) ) ;
#42488=CARTESIAN_POINT ( 'NONE',  ( -1.050000000000037792, 2.500000000000000000, 1.918653347947321564 ) ) ;
#42489=DIRECTION ( 'NONE',  ( 0.000000000000000000, 0.000000000000000000, -1.000000000000000000 ) ) ;
#42490=VECTOR ( 'NONE', #15080, 1000.000000000000000 ) ;
#42491=CONICAL_SURFACE ( 'NONE', #40342, 0.09999999999999999167, 0.003490658503988666988 ) ;
#42493=AXIS2_PLACEMENT_3D ( 'NONE', #59042, #108764, #49237 ) ;
#42494=VERTEX_POINT ( 'NONE', #121689 ) ;
#42495=ORIENTED_EDGE ( 'NONE', *, *, #119006, .F. ) ;
#42496=CARTESIAN_POINT ( 'NONE',  ( -11.44999999999999751, 12.50000000000000000, -2.446380397790836270 ) ) ;
#42497=FACE_OUTER_BOUND ( 'NONE', #46220, .T. ) ;
#42498=DIRECTION ( 'NONE',  ( 0.000000000000000000, 0.000000000000000000, -1.000000000000000000 ) ) ;
#42499=FACE_BOUND ( 'NONE', #97956, .T. ) ;
#42500=DIRECTION ( 'NONE',  ( 0.000000000000000000, 0.000000000000000000, 1.000000000000000000 ) ) ;
#42501=AXIS2_PLACEMENT_3D ( 'NONE', #14563, #42783, #53229 ) ;
#42502=CARTESIAN_POINT ( 'NONE',  ( 5.449999999999937117, 2.500000000000000000, -6.595190528383302109 ) ) ;
#42503=ADVANCED_FACE ( 'NONE', ( #91595 ), #92949, .T. ) ;
#42504=DIRECTION ( 'NONE',  ( 0.000000000000000000, 0.000000000000000000, -1.000000000000000000 ) ) ;
#42505=AXIS2_PLACEMENT_3D ( 'NONE', #102375, #93202, #53913 ) ;
#42506=AXIS2_PLACEMENT_3D ( 'NONE', #28428, #9425, #97159 ) ;
#42507=AXIS2_PLACEMENT_3D ( 'NONE', #31931, #1804, #100025 ) ;
#42508=EDGE_CURVE ( 'NONE', #92907, #15629, #113870, .T. ) ;
#42509=EDGE_CURVE ( 'NONE', #54541, #21011, #107607, .T. ) ;
#42510=CARTESIAN_POINT ( 'NONE',  ( -0.4500000000000397571, 2.500000000000000000, -6.495190528383302464 ) ) ;
#42512=AXIS2_PLACEMENT_3D ( 'NONE', #112385, #122842, #23334 ) ;
#42513=EDGE_CURVE ( 'NONE', #129360, #94388, #124335, .T. ) ;
#42514=CARTESIAN_POINT ( 'NONE',  ( 8.149999999999920419, 12.50000000000000000, 6.841600689897072485 ) ) ;
#42515=ORIENTED_EDGE ( 'NONE', *, *, #86935, .F. ) ;
#42516=ADVANCED_FACE ( 'NONE', ( #22229 ), #67882, .T. ) ;
#42517=DIRECTION ( 'NONE',  ( 0.000000000000000000, 0.000000000000000000, 1.000000000000000000 ) ) ;
#42518=DIRECTION ( 'NONE',  ( 0.000000000000000000, 1.000000000000000000, 0.000000000000000000 ) ) ;
#42519=AXIS2_PLACEMENT_3D ( 'NONE', #5003, #123492, #75051 ) ;
#42520=ADVANCED_FACE ( 'NONE', ( #122359 ), #90953, .T. ) ;
#42522=EDGE_LOOP ( 'NONE', ( #44760, #8526 ) ) ;
#42523=CARTESIAN_POINT ( 'NONE',  ( 8.349999999999923261, 2.500000000000000000, -7.088010851410853519 ) ) ;
#42524=DIRECTION ( 'NONE',  ( 0.000000000000000000, 0.000000000000000000, 1.000000000000000000 ) ) ;
#42525=FACE_BOUND ( 'NONE', #114536, .T. ) ;
#42526=CARTESIAN_POINT ( 'NONE',  ( -2.100000000000033396, 2.500000000000000000, -3.637306695894650055 ) ) ;
#42527=EDGE_CURVE ( 'NONE', #23084, #125100, #26137, .T. ) ;
#42528=ADVANCED_FACE ( 'NONE', ( #1277 ), #101357, .T. ) ;
#42529=CONICAL_SURFACE ( 'NONE', #734, 0.1000000000000002554, 0.003490658503988666988 ) ;
#42530=ORIENTED_EDGE ( 'NONE', *, *, #52511, .F. ) ;
#42531=CARTESIAN_POINT ( 'NONE',  ( 10.59999999999990905, 2.500000000000000000, 3.883716857408420431 ) ) ;
#42532=CIRCLE ( 'NONE', #75946, 0.06509327318403745899 ) ;
#42533=DIRECTION ( 'NONE',  ( 0.000000000000000000, 0.000000000000000000, 1.000000000000000000 ) ) ;
#42534=ORIENTED_EDGE ( 'NONE', *, *, #115326, .T. ) ;
#42535=DIRECTION ( 'NONE',  ( -4.274815082592931898E-19, -0.9999939076577903929, -0.003490651415223739937 ) ) ;
#42536=FACE_OUTER_BOUND ( 'NONE', #6263, .T. ) ;
#42537=CIRCLE ( 'NONE', #126137, 0.1000000000000002554 ) ;
#42538=CONICAL_SURFACE ( 'NONE', #84373, 0.09999999999999982514, 0.003490658503988666988 ) ;
#42539=CIRCLE ( 'NONE', #96884, 0.06509327318403745899 ) ;
#42540=AXIS2_PLACEMENT_3D ( 'NONE', #108896, #107628, #18601 ) ;
#42541=ORIENTED_EDGE ( 'NONE', *, *, #54314, .T. ) ;
#42542=DIRECTION ( 'NONE',  ( 0.000000000000000000, 1.000000000000000000, 0.000000000000000000 ) ) ;
#42543=CARTESIAN_POINT ( 'NONE',  ( -7.050000000000013145, 2.500000000000000000, 6.495190528383297135 ) ) ;
#42544=EDGE_CURVE ( 'NONE', #29211, #97516, #95091, .T. ) ;
#42545=CIRCLE ( 'NONE', #48797, 0.06509327318403745899 ) ;
#42546=ORIENTED_EDGE ( 'NONE', *, *, #13062, .F. ) ;
#42547=DIRECTION ( 'NONE',  ( 0.000000000000000000, -0.9999939076577903929, 0.003490651415223739937 ) ) ;
#42548=CARTESIAN_POINT ( 'NONE',  ( 5.649999999999936406, 2.500000000000000000, -6.048780366869526581 ) ) ;
#42549=CARTESIAN_POINT ( 'NONE',  ( -6.850000000000013856, 2.500000000000000000, 6.841600689897072485 ) ) ;
#42550=VECTOR ( 'NONE', #45626, 1000.000000000000000 ) ;
#42551=VECTOR ( 'NONE', #102152, 1000.000000000000000 ) ;
#42552=ORIENTED_EDGE ( 'NONE', *, *, #39262, .F. ) ;
#42553=ORIENTED_EDGE ( 'NONE', *, *, #51387, .F. ) ;
#42554=CARTESIAN_POINT ( 'NONE',  ( -0.8000000000000315747, 2.500000000000000000, 0.1000000000000000056 ) ) ;
#42555=ORIENTED_EDGE ( 'NONE', *, *, #26963, .T. ) ;
#42556=CARTESIAN_POINT ( 'NONE',  ( 8.749999999999953815, 2.500000000000000000, 6.395190528383296602 ) ) ;
#42557=DIRECTION ( 'NONE',  ( 0.000000000000000000, 0.000000000000000000, -1.000000000000000000 ) ) ;
#42558=DIRECTION ( 'NONE',  ( 0.000000000000000000, -0.000000000000000000, 1.000000000000000000 ) ) ;
#42559=ORIENTED_EDGE ( 'NONE', *, *, #38518, .T. ) ;
#42560=FACE_OUTER_BOUND ( 'NONE', #66766, .T. ) ;
#42561=CARTESIAN_POINT ( 'NONE',  ( 5.449999999999937117, 12.50000000000000000, -6.560283801567339701 ) ) ;
#42562=CARTESIAN_POINT ( 'NONE',  ( -14.14999999999998614, 2.500000000000000000, 1.472243186433549456 ) ) ;
#42564=DIRECTION ( 'NONE',  ( -0.000000000000000000, -1.000000000000000000, -0.000000000000000000 ) ) ;
#42565=DIRECTION ( 'NONE',  ( 0.000000000000000000, 0.000000000000000000, 1.000000000000000000 ) ) ;
#42566=DIRECTION ( 'NONE',  ( 0.000000000000000000, 0.000000000000000000, -1.000000000000000000 ) ) ;
#42568=ORIENTED_EDGE ( 'NONE', *, *, #98971, .T. ) ;
#42569=EDGE_CURVE ( 'NONE', #45906, #126243, #31401, .T. ) ;
#42570=ORIENTED_EDGE ( 'NONE', *, *, #5669, .F. ) ;
#42571=DIRECTION ( 'NONE',  ( 0.000000000000000000, 0.000000000000000000, -1.000000000000000000 ) ) ;
#42572=VERTEX_POINT ( 'NONE', #52316 ) ;
#42573=DIRECTION ( 'NONE',  ( -4.274815082592931898E-19, -0.9999939076577903929, -0.003490651415223739937 ) ) ;
#42574=EDGE_LOOP ( 'NONE', ( #20325, #72969 ) ) ;
#42575=ORIENTED_EDGE ( 'NONE', *, *, #76862, .T. ) ;
#42576=ORIENTED_EDGE ( 'NONE', *, *, #24774, .F. ) ;
#42577=DIRECTION ( 'NONE',  ( 0.000000000000000000, 0.000000000000000000, -1.000000000000000000 ) ) ;
#42578=AXIS2_PLACEMENT_3D ( 'NONE', #11269, #71474, #121228 ) ;
#42579=DIRECTION ( 'NONE',  ( 0.000000000000000000, 0.000000000000000000, 1.000000000000000000 ) ) ;
#42580=VECTOR ( 'NONE', #45552, 1000.000000000000000 ) ;
#42581=CARTESIAN_POINT ( 'NONE',  ( 4.149999999999941735, 2.500000000000000000, -5.802370205355749988 ) ) ;
#42582=DIRECTION ( 'NONE',  ( 0.000000000000000000, 1.000000000000000000, 0.000000000000000000 ) ) ;
#42583=CARTESIAN_POINT ( 'NONE',  ( -1.050000000000037348, 12.50000000000000000, -2.576566944158915184 ) ) ;
#42584=DIRECTION ( 'NONE',  ( -0.000000000000000000, 1.000000000000000000, -0.000000000000000000 ) ) ;
#42585=CARTESIAN_POINT ( 'NONE',  ( 11.64999999999990621, 2.500000000000000000, 6.495190528383297135 ) ) ;
#42586=DIRECTION ( 'NONE',  ( -0.000000000000000000, -1.000000000000000000, -0.000000000000000000 ) ) ;
#42587=AXIS2_PLACEMENT_3D ( 'NONE', #15593, #45723, #104621 ) ;
#42588=AXIS2_PLACEMENT_3D ( 'NONE', #5545, #55941, #43570 ) ;
#42589=DIRECTION ( 'NONE',  ( 0.000000000000000000, 0.000000000000000000, 1.000000000000000000 ) ) ;
#42590=AXIS2_PLACEMENT_3D ( 'NONE', #61224, #348, #52056 ) ;
#42592=VECTOR ( 'NONE', #101540, 1000.000000000000000 ) ;
#42593=DIRECTION ( 'NONE',  ( 0.000000000000000000, -0.9999939076577903929, 0.003490651415223739937 ) ) ;
#42594=ORIENTED_EDGE ( 'NONE', *, *, #71720, .F. ) ;
#42595=ORIENTED_EDGE ( 'NONE', *, *, #13362, .F. ) ;
#42596=DIRECTION ( 'NONE',  ( -0.000000000000000000, -1.000000000000000000, -0.000000000000000000 ) ) ;
#42597=DIRECTION ( 'NONE',  ( -0.000000000000000000, 1.000000000000000000, -0.000000000000000000 ) ) ;
#42598=AXIS2_PLACEMENT_3D ( 'NONE', #54748, #105142, #25282 ) ;
#42599=DIRECTION ( 'NONE',  ( 0.000000000000000000, -0.9999939076577903929, 0.003490651415223739937 ) ) ;
#42600=CARTESIAN_POINT ( 'NONE',  ( -5.600000000000020073, 12.50000000000000000, 4.676537180435972552 ) ) ;
#42601=DIRECTION ( 'NONE',  ( 0.000000000000000000, 0.000000000000000000, 1.000000000000000000 ) ) ;
#42602=CONICAL_SURFACE ( 'NONE', #113686, 0.09999999999999982514, 0.003490658503988666988 ) ;
#42604=CIRCLE ( 'NONE', #19597, 0.06509327318403745899 ) ;
#42605=DIRECTION ( 'NONE',  ( 0.000000000000000000, 1.000000000000000000, 0.000000000000000000 ) ) ;
#42606=EDGE_LOOP ( 'NONE', ( #91113, #14487 ) ) ;
#42607=VECTOR ( 'NONE', #29799, 1000.000000000000000 ) ;
#42608=CIRCLE ( 'NONE', #19605, 0.06509327318403745899 ) ;
#42609=ORIENTED_EDGE ( 'NONE', *, *, #28324, .T. ) ;
#42610=EDGE_CURVE ( 'NONE', #112676, #45445, #20924, .T. ) ;
#42611=EDGE_LOOP ( 'NONE', ( #76697, #126730 ) ) ;
#42612=ORIENTED_EDGE ( 'NONE', *, *, #5528, .T. ) ;
#42613=ADVANCED_FACE ( 'NONE', ( #71298 ), #109666, .T. ) ;
#42614=ORIENTED_EDGE ( 'NONE', *, *, #118237, .T. ) ;
#42615=ADVANCED_FACE ( 'NONE', ( #24631 ), #53241, .T. ) ;
#42616=FACE_OUTER_BOUND ( 'NONE', #60655, .T. ) ;
#42617=PLANE ( 'NONE',  #122955 ) ;
#42618=CARTESIAN_POINT ( 'NONE',  ( -6.071532165918824830E-15, 2.500000000000000000, -4.330127018922201643 ) ) ;
#42619=DIRECTION ( 'NONE',  ( 0.000000000000000000, -0.000000000000000000, 1.000000000000000000 ) ) ;
#42620=ADVANCED_FACE ( 'NONE', ( #66473 ), #63703, .T. ) ;
#42621=CARTESIAN_POINT ( 'NONE',  ( 3.099999999999945466, 2.500000000000000000, -3.983716857408426293 ) ) ;
#42623=ORIENTED_EDGE ( 'NONE', *, *, #95989, .F. ) ;
#42624=CARTESIAN_POINT ( 'NONE',  ( 5.199999999999931788, 12.50000000000000000, 4.741630453620009789 ) ) ;
#42625=VECTOR ( 'NONE', #91510, 1000.000000000000000 ) ;
#42626=EDGE_CURVE ( 'NONE', #98546, #54633, #16068, .T. ) ;
#42627=DIRECTION ( 'NONE',  ( 0.000000000000000000, 0.000000000000000000, 1.000000000000000000 ) ) ;
#42628=ADVANCED_FACE ( 'NONE', ( #96565 ), #22032, .T. ) ;
#42629=DIRECTION ( 'NONE',  ( 0.000000000000000000, 0.000000000000000000, 1.000000000000000000 ) ) ;
#42630=DIRECTION ( 'NONE',  ( 0.000000000000000000, 0.000000000000000000, -1.000000000000000000 ) ) ;
#42631=EDGE_LOOP ( 'NONE', ( #17043, #120365 ) ) ;
#42632=CONICAL_SURFACE ( 'NONE', #67634, 0.1000000000000000472, 0.003490658503988666988 ) ;
#42633=CIRCLE ( 'NONE', #61501, 0.1000000000000000472 ) ;
#42634=AXIS2_PLACEMENT_3D ( 'NONE', #42136, #70948, #1552 ) ;
#42635=ORIENTED_EDGE ( 'NONE', *, *, #109961, .T. ) ;
#42636=AXIS2_PLACEMENT_3D ( 'NONE', #87451, #10198, #9557 ) ;
#42637=EDGE_LOOP ( 'NONE', ( #42866, #99781, #6600, #56266 ) ) ;
#42638=CONICAL_SURFACE ( 'NONE', #59364, 0.09999999999999999167, 0.003490658503988666988 ) ;
#42639=LINE ( 'NONE', #101538, #101105 ) ;
#42641=ORIENTED_EDGE ( 'NONE', *, *, #116746, .T. ) ;
#42642=CARTESIAN_POINT ( 'NONE',  ( 5.449999999999936229, 2.500000000000000000, -2.165063509461101710 ) ) ;
#42643=CARTESIAN_POINT ( 'NONE',  ( -2.500000000000031086, 2.500000000000000000, 3.537306695894645081 ) ) ;
#42644=AXIS2_PLACEMENT_3D ( 'NONE', #96855, #117128, #67366 ) ;
#42645=AXIS2_PLACEMENT_3D ( 'NONE', #46430, #64142, #53686 ) ;
#42646=AXIS2_PLACEMENT_3D ( 'NONE', #125874, #36234, #7389 ) ;
#42647=CIRCLE ( 'NONE', #115775, 0.09999999999999982514 ) ;
#42648=ORIENTED_EDGE ( 'NONE', *, *, #47946, .T. ) ;
#42649=FACE_OUTER_BOUND ( 'NONE', #78449, .T. ) ;
#42650=DIRECTION ( 'NONE',  ( 0.000000000000000000, -0.9999939076577903929, 0.003490651415223739937 ) ) ;
#42651=CARTESIAN_POINT ( 'NONE',  ( -8.550000000000013145, 12.50000000000000000, -1.818653347947326138 ) ) ;
#42652=CARTESIAN_POINT ( 'NONE',  ( -0.8500000000000395017, 2.500000000000000000, 2.065063509461097624 ) ) ;
#42653=CARTESIAN_POINT ( 'NONE',  ( -8.950000000000011724, 2.500000000000000000, -6.148780366869520897 ) ) ;
#42654=VERTEX_POINT ( 'NONE', #55377 ) ;
#42655=ORIENTED_EDGE ( 'NONE', *, *, #37156, .F. ) ;
#42656=EDGE_CURVE ( 'NONE', #11179, #9679, #75639, .T. ) ;
#42658=LINE ( 'NONE', #32194, #12167 ) ;
#42659=LINE ( 'NONE', #94297, #86840 ) ;
#42660=CIRCLE ( 'NONE', #44798, 0.1000000000000000472 ) ;
#42661=DIRECTION ( 'NONE',  ( 0.000000000000000000, 0.000000000000000000, 1.000000000000000000 ) ) ;
#42662=ORIENTED_EDGE ( 'NONE', *, *, #24579, .T. ) ;
#42663=ORIENTED_EDGE ( 'NONE', *, *, #14564, .F. ) ;
#42664=EDGE_CURVE ( 'NONE', #29584, #93873, #97869, .T. ) ;
#42665=CARTESIAN_POINT ( 'NONE',  ( 4.149999999999939959, 2.500000000000000000, 2.957883832488649389 ) ) ;
#42666=DIRECTION ( 'NONE',  ( 0.000000000000000000, 0.000000000000000000, -1.000000000000000000 ) ) ;
#42667=CARTESIAN_POINT ( 'NONE',  ( -11.84999999999999609, 12.50000000000000000, 6.148780366869520897 ) ) ;
#42668=ADVANCED_FACE ( 'NONE', ( #115558 ), #105102, .T. ) ;
#42669=LINE ( 'NONE', #113964, #88619 ) ;
#42670=ORIENTED_EDGE ( 'NONE', *, *, #29390, .T. ) ;
#42671=AXIS2_PLACEMENT_3D ( 'NONE', #50252, #40446, #30624 ) ;
#42672=CIRCLE ( 'NONE', #78166, 0.1000000000000002554 ) ;
#42673=CARTESIAN_POINT ( 'NONE',  ( 0.3999999999999628852, 12.50000000000000000, 0.6928203230275518099 ) ) ;
#42674=ADVANCED_FACE ( 'NONE', ( #106402 ), #59703, .T. ) ;
#42675=DIRECTION ( 'NONE',  ( -0.000000000000000000, 1.000000000000000000, -0.000000000000000000 ) ) ;
#42676=ORIENTED_EDGE ( 'NONE', *, *, #45035, .F. ) ;
#42677=DIRECTION ( 'NONE',  ( 0.000000000000000000, -0.9999939076577903929, 0.003490651415223739937 ) ) ;
#42678=EDGE_CURVE ( 'NONE', #43625, #116926, #6885, .T. ) ;
#42679=AXIS2_PLACEMENT_3D ( 'NONE', #50870, #121522, #53456 ) ;
#42680=ORIENTED_EDGE ( 'NONE', *, *, #18548, .F. ) ;
#42681=DIRECTION ( 'NONE',  ( 0.000000000000000000, -0.9999939076577903929, 0.003490651415223739937 ) ) ;
#42682=EDGE_CURVE ( 'NONE', #122820, #122810, #88922, .T. ) ;
#42683=AXIS2_PLACEMENT_3D ( 'NONE', #95195, #5502, #113539 ) ;
#42684=ADVANCED_FACE ( 'NONE', ( #126031 ), #49231, .T. ) ;
#42685=EDGE_CURVE ( 'NONE', #120064, #14553, #38774, .T. ) ;
#42686=ORIENTED_EDGE ( 'NONE', *, *, #69846, .T. ) ;
#42687=FACE_OUTER_BOUND ( 'NONE', #19806, .T. ) ;
#42688=DIRECTION ( 'NONE',  ( 0.000000000000000000, 0.000000000000000000, 1.000000000000000000 ) ) ;
#42689=VERTEX_POINT ( 'NONE', #86757 ) ;
#42690=VERTEX_POINT ( 'NONE', #36397 ) ;
#42692=DIRECTION ( 'NONE',  ( 0.000000000000000000, -0.000000000000000000, 1.000000000000000000 ) ) ;
#42693=EDGE_CURVE ( 'NONE', #61962, #97794, #51290, .T. ) ;
#42696=VECTOR ( 'NONE', #121199, 1000.000000000000000 ) ;
#42697=CARTESIAN_POINT ( 'NONE',  ( 0.3999999999999563904, 2.500000000000000000, 3.637306695894644726 ) ) ;
#42698=CONICAL_SURFACE ( 'NONE', #99118, 0.09999999999999982514, 0.003490658503988666988 ) ;
#42699=AXIS2_PLACEMENT_3D ( 'NONE', #38822, #8653, #66935 ) ;
#42700=CARTESIAN_POINT ( 'NONE',  ( -1.250000000000001554, 2.500000000000000000, 6.495190528383297135 ) ) ;
#42701=DIRECTION ( 'NONE',  ( 0.000000000000000000, -0.000000000000000000, 1.000000000000000000 ) ) ;
#42702=LINE ( 'NONE', #30937, #39031 ) ;
#42703=VECTOR ( 'NONE', #88552, 1000.000000000000000 ) ;
#42704=PLANE ( 'NONE',  #123673 ) ;
#42705=AXIS2_PLACEMENT_3D ( 'NONE', #101249, #41705, #11574 ) ;
#42706=ORIENTED_EDGE ( 'NONE', *, *, #79572, .T. ) ;
#42707=ORIENTED_EDGE ( 'NONE', *, *, #32582, .F. ) ;
#42708=FACE_OUTER_BOUND ( 'NONE', #7312, .T. ) ;
#42709=EDGE_LOOP ( 'NONE', ( #95631, #85727 ) ) ;
#42710=DIRECTION ( 'NONE',  ( -4.274815082592931898E-19, -0.9999939076577903929, -0.003490651415223739937 ) ) ;
#42711=CARTESIAN_POINT ( 'NONE',  ( 7.499999999999925393, 2.500000000000000000, -3.537306695894649966 ) ) ;
#42712=DIRECTION ( 'NONE',  ( -0.000000000000000000, 1.000000000000000000, -0.000000000000000000 ) ) ;
#42713=ORIENTED_EDGE ( 'NONE', *, *, #45298, .F. ) ;
#42714=ORIENTED_EDGE ( 'NONE', *, *, #124308, .T. ) ;
#42715=FACE_BOUND ( 'NONE', #99298, .T. ) ;
#42716=ORIENTED_EDGE ( 'NONE', *, *, #101863, .F. ) ;
#42717=CARTESIAN_POINT ( 'NONE',  ( 11.89999999999990798, 12.50000000000000000, 3.983716857408420964 ) ) ;
#42718=CARTESIAN_POINT ( 'NONE',  ( -0.4000000000000331624, 2.500000000000000000, -0.6928203230275519209 ) ) ;
#42719=DIRECTION ( 'NONE',  ( 0.000000000000000000, 0.000000000000000000, 1.000000000000000000 ) ) ;
#42720=DIRECTION ( 'NONE',  ( 0.000000000000000000, 0.000000000000000000, 1.000000000000000000 ) ) ;
#42721=DIRECTION ( 'NONE',  ( 0.000000000000000000, -0.9999939076577903929, 0.003490651415223739937 ) ) ;
#42722=CARTESIAN_POINT ( 'NONE',  ( -10.84999999999999964, 2.500000000000000000, 7.188010851410848723 ) ) ;
#42723=AXIS2_PLACEMENT_3D ( 'NONE', #44348, #82369, #62079 ) ;
#42724=DIRECTION ( 'NONE',  ( 0.000000000000000000, 1.000000000000000000, 0.000000000000000000 ) ) ;
#42725=DIRECTION ( 'NONE',  ( 0.000000000000000000, 1.000000000000000000, 0.000000000000000000 ) ) ;
#42726=AXIS2_PLACEMENT_3D ( 'NONE', #97947, #118235, #8271 ) ;
#42727=AXIS2_PLACEMENT_3D ( 'NONE', #85516, #123498, #94051 ) ;
#42728=DIRECTION ( 'NONE',  ( 0.000000000000000000, 1.000000000000000000, 0.000000000000000000 ) ) ;
#42729=DIRECTION ( 'NONE',  ( -4.274815082592931898E-19, -0.9999939076577903929, -0.003490651415223739937 ) ) ;
#42730=DIRECTION ( 'NONE',  ( 0.000000000000000000, 1.000000000000000000, 0.000000000000000000 ) ) ;
#42731=CIRCLE ( 'NONE', #76152, 0.06509327318403745899 ) ;
#42732=VECTOR ( 'NONE', #120198, 1000.000000000000000 ) ;
#42733=VERTEX_POINT ( 'NONE', #67091 ) ;
#42734=VERTEX_POINT ( 'NONE', #107032 ) ;
#42735=ADVANCED_FACE ( 'NONE', ( #17357 ), #57313, .T. ) ;
#42736=EDGE_LOOP ( 'NONE', ( #48502, #83314, #115458, #40406 ) ) ;
#42737=AXIS2_PLACEMENT_3D ( 'NONE', #102460, #43556, #50783 ) ;
#42738=CARTESIAN_POINT ( 'NONE',  ( -1.900000000000034106, 12.50000000000000000, 0.3464101615137735735 ) ) ;
#42739=ORIENTED_EDGE ( 'NONE', *, *, #37873, .F. ) ;
#42740=DIRECTION ( 'NONE',  ( 0.000000000000000000, 0.000000000000000000, 1.000000000000000000 ) ) ;
#42741=VERTEX_POINT ( 'NONE', #68405 ) ;
#42742=ORIENTED_EDGE ( 'NONE', *, *, #5274, .T. ) ;
#42744=CARTESIAN_POINT ( 'NONE',  ( -7.900000000000014566, 12.50000000000000000, -4.957854068765716882 ) ) ;
#42745=CONICAL_SURFACE ( 'NONE', #90534, 0.1000000000000002554, 0.003490658503988666988 ) ;
#42746=AXIS2_PLACEMENT_3D ( 'NONE', #35341, #25493, #85711 ) ;
#42747=CIRCLE ( 'NONE', #57290, 0.1000000000000002554 ) ;
#42748=CARTESIAN_POINT ( 'NONE',  ( 9.999999999999952038, 12.50000000000000000, -0.06509327318403970719 ) ) ;
#42749=DIRECTION ( 'NONE',  ( -0.000000000000000000, 1.000000000000000000, -0.000000000000000000 ) ) ;
#42750=CARTESIAN_POINT ( 'NONE',  ( 21.24754738303276724, -0.7337760880902383098, -4.182111650399352953 ) ) ;
#42751=DIRECTION ( 'NONE',  ( -0.000000000000000000, -1.000000000000000000, -0.000000000000000000 ) ) ;
#42752=VECTOR ( 'NONE', #39240, 1000.000000000000000 ) ;
#42753=DIRECTION ( 'NONE',  ( 0.000000000000000000, 0.000000000000000000, 1.000000000000000000 ) ) ;
#42754=EDGE_CURVE ( 'NONE', #28650, #66463, #29779, .T. ) ;
#42755=VERTEX_POINT ( 'NONE', #69703 ) ;
#42756=DIRECTION ( 'NONE',  ( 0.000000000000000000, 0.000000000000000000, -1.000000000000000000 ) ) ;
#42757=VERTEX_POINT ( 'NONE', #98500 ) ;
#42758=ORIENTED_EDGE ( 'NONE', *, *, #30480, .T. ) ;
#42759=ORIENTED_EDGE ( 'NONE', *, *, #122854, .F. ) ;
#42761=EDGE_LOOP ( 'NONE', ( #36358, #63161 ) ) ;
#42762=EDGE_LOOP ( 'NONE', ( #103215, #80588 ) ) ;
#42763=ORIENTED_EDGE ( 'NONE', *, *, #121071, .F. ) ;
#42764=CIRCLE ( 'NONE', #113839, 0.1000000000000002554 ) ;
#42766=DIRECTION ( 'NONE',  ( 0.000000000000000000, 1.000000000000000000, 0.000000000000000000 ) ) ;
#42767=DIRECTION ( 'NONE',  ( 0.000000000000000000, 1.000000000000000000, 0.000000000000000000 ) ) ;
#42769=CARTESIAN_POINT ( 'NONE',  ( 0.3999999999999628852, 2.500000000000000000, 0.6928203230275518099 ) ) ;
#42770=CARTESIAN_POINT ( 'NONE',  ( 5.399999999999931966, 2.500000000000000000, 4.430127018922196847 ) ) ;
#42771=DIRECTION ( 'NONE',  ( 0.000000000000000000, 0.000000000000000000, 1.000000000000000000 ) ) ;
#42772=CIRCLE ( 'NONE', #11433, 0.06509327318403745899 ) ;
#42773=CIRCLE ( 'NONE', #115891, 0.1000000000000002554 ) ;
#42775=DIRECTION ( 'NONE',  ( -4.274815082592931898E-19, -0.9999939076577903929, -0.003490651415223739937 ) ) ;
#42776=EDGE_CURVE ( 'NONE', #129065, #100019, #10750, .T. ) ;
#42777=EDGE_LOOP ( 'NONE', ( #42739, #78610 ) ) ;
#42778=CARTESIAN_POINT ( 'NONE',  ( -6.249999999999981348, 12.50000000000000000, 2.165063509461097713 ) ) ;
#42779=VERTEX_POINT ( 'NONE', #21241 ) ;
#42780=FACE_OUTER_BOUND ( 'NONE', #39101, .T. ) ;
#42781=VERTEX_POINT ( 'NONE', #50706 ) ;
#42782=EDGE_CURVE ( 'NONE', #97955, #24335, #76307, .T. ) ;
#42783=DIRECTION ( 'NONE',  ( -0.000000000000000000, -1.000000000000000000, -0.000000000000000000 ) ) ;
#42784=AXIS2_PLACEMENT_3D ( 'NONE', #72899, #63726, #84648 ) ;
#42785=DIRECTION ( 'NONE',  ( 0.000000000000000000, -0.000000000000000000, 1.000000000000000000 ) ) ;
#42786=ORIENTED_EDGE ( 'NONE', *, *, #9792, .T. ) ;
#42787=EDGE_CURVE ( 'NONE', #57274, #38043, #9500, .T. ) ;
#42788=ADVANCED_FACE ( 'NONE', ( #18669 ), #57532, .T. ) ;
#42789=ORIENTED_EDGE ( 'NONE', *, *, #7789, .F. ) ;
#42790=DIRECTION ( 'NONE',  ( 0.000000000000000000, 0.000000000000000000, 1.000000000000000000 ) ) ;
#42792=ADVANCED_FACE ( 'NONE', ( #19967 ), #8833, .T. ) ;
#42793=DIRECTION ( 'NONE',  ( -0.000000000000000000, -1.000000000000000000, -0.000000000000000000 ) ) ;
#42794=EDGE_CURVE ( 'NONE', #111573, #116963, #28286, .T. ) ;
#42795=ADVANCED_FACE ( 'NONE', ( #119434 ), #61175, .T. ) ;
#42796=CARTESIAN_POINT ( 'NONE',  ( 6.049999999999932321, 2.500000000000000000, 6.941600689897073018 ) ) ;
#42797=DIRECTION ( 'NONE',  ( 0.000000000000000000, 0.000000000000000000, 1.000000000000000000 ) ) ;
#42798=ORIENTED_EDGE ( 'NONE', *, *, #124733, .F. ) ;
#42799=AXIS2_PLACEMENT_3D ( 'NONE', #21061, #42004, #12529 ) ;
#42800=CARTESIAN_POINT ( 'NONE',  ( 4.149999999999939959, 2.500000000000000000, 2.857883832488649301 ) ) ;
#42801=AXIS2_PLACEMENT_3D ( 'NONE', #4031, #24333, #103546 ) ;
#42802=EDGE_CURVE ( 'NONE', #128741, #31897, #19880, .T. ) ;
#42803=ORIENTED_EDGE ( 'NONE', *, *, #79038, .T. ) ;
#42805=DIRECTION ( 'NONE',  ( 0.000000000000000000, -0.000000000000000000, 1.000000000000000000 ) ) ;
#42806=CARTESIAN_POINT ( 'NONE',  ( -9.350000000000004974, 2.500000000000000000, 6.841600689897072485 ) ) ;
#42807=EDGE_CURVE ( 'NONE', #76002, #127039, #66500, .T. ) ;
#42809=CARTESIAN_POINT ( 'NONE',  ( 8.549999999999920774, 2.500000000000000000, -2.411473670974877859 ) ) ;
#42810=CARTESIAN_POINT ( 'NONE',  ( -4.350000000000023626, 12.50000000000000000, 6.148780366869520897 ) ) ;
#42811=DIRECTION ( 'NONE',  ( -0.000000000000000000, -1.000000000000000000, -0.000000000000000000 ) ) ;
#42812=DIRECTION ( 'NONE',  ( 0.000000000000000000, 0.000000000000000000, 1.000000000000000000 ) ) ;
#42813=ORIENTED_EDGE ( 'NONE', *, *, #59498, .T. ) ;
#42814=DIRECTION ( 'NONE',  ( -0.000000000000000000, 1.000000000000000000, -0.000000000000000000 ) ) ;
#42815=AXIS2_PLACEMENT_3D ( 'NONE', #119684, #118402, #119059 ) ;
#42816=DIRECTION ( 'NONE',  ( -0.000000000000000000, -0.000000000000000000, -1.000000000000000000 ) ) ;
#42817=CARTESIAN_POINT ( 'NONE',  ( 12.09999999999990550, 12.50000000000000000, 5.022947341949748790 ) ) ;
#42818=CIRCLE ( 'NONE', #26063, 0.09999999999999982514 ) ;
#42819=ORIENTED_EDGE ( 'NONE', *, *, #42942, .F. ) ;
#42820=VECTOR ( 'NONE', #126627, 1000.000000000000000 ) ;
#42821=AXIS2_PLACEMENT_3D ( 'NONE', #17400, #57348, #28538 ) ;
#42822=DIRECTION ( 'NONE',  ( -0.000000000000000000, -1.000000000000000000, -0.000000000000000000 ) ) ;
#42823=CIRCLE ( 'NONE', #115949, 0.06509327318403745899 ) ;
#42824=AXIS2_PLACEMENT_3D ( 'NONE', #41904, #122393, #112573 ) ;
#42825=VERTEX_POINT ( 'NONE', #89350 ) ;
#42826=VECTOR ( 'NONE', #78164, 1000.000000000000000 ) ;
#42827=ORIENTED_EDGE ( 'NONE', *, *, #75287, .F. ) ;
#42828=DIRECTION ( 'NONE',  ( -0.000000000000000000, 1.000000000000000000, -0.000000000000000000 ) ) ;
#42830=EDGE_LOOP ( 'NONE', ( #100711, #115635, #48048, #119923 ) ) ;
#42831=CARTESIAN_POINT ( 'NONE',  ( -5.600000000000020073, 2.500000000000000000, 0.2464101615137736789 ) ) ;
#42832=DIRECTION ( 'NONE',  ( 0.000000000000000000, 0.000000000000000000, 1.000000000000000000 ) ) ;
#42833=DIRECTION ( 'NONE',  ( -4.274815082592931898E-19, -0.9999939076577903929, -0.003490651415223739937 ) ) ;
#42834=EDGE_LOOP ( 'NONE', ( #76133, #87431 ) ) ;
#42835=CIRCLE ( 'NONE', #30301, 0.09999999999999982514 ) ;
#42836=AXIS2_PLACEMENT_3D ( 'NONE', #47679, #7727, #31110 ) ;
#42837=DIRECTION ( 'NONE',  ( 0.000000000000000000, 0.000000000000000000, 1.000000000000000000 ) ) ;
#42838=CARTESIAN_POINT ( 'NONE',  ( 10.19999999999991402, 12.50000000000000000, 0.3464101615137735735 ) ) ;
#42839=VECTOR ( 'NONE', #120838, 1000.000000000000000 ) ;
#42840=EDGE_CURVE ( 'NONE', #51134, #65511, #70350, .T. ) ;
#42841=ORIENTED_EDGE ( 'NONE', *, *, #121527, .F. ) ;
#42842=EDGE_CURVE ( 'NONE', #115296, #123777, #13594, .T. ) ;
#42843=ORIENTED_EDGE ( 'NONE', *, *, #44111, .T. ) ;
#42844=ADVANCED_FACE ( 'NONE', ( #39632 ), #72208, .T. ) ;
#42845=EDGE_LOOP ( 'NONE', ( #66251, #42416, #39914, #32661 ) ) ;
#42846=FACE_OUTER_BOUND ( 'NONE', #2184, .T. ) ;
#42847=FACE_OUTER_BOUND ( 'NONE', #38561, .T. ) ;
#42848=DIRECTION ( 'NONE',  ( 0.000000000000000000, -0.9999939076577903929, 0.003490651415223739937 ) ) ;
#42849=FACE_BOUND ( 'NONE', #40566, .T. ) ;
#42850=VERTEX_POINT ( 'NONE', #50093 ) ;
#42851=DIRECTION ( 'NONE',  ( 0.000000000000000000, 0.000000000000000000, -1.000000000000000000 ) ) ;
#42852=DIRECTION ( 'NONE',  ( 0.000000000000000000, 0.000000000000000000, 1.000000000000000000 ) ) ;
#42853=CIRCLE ( 'NONE', #57405, 0.1000000000000002554 ) ;
#42854=ORIENTED_EDGE ( 'NONE', *, *, #117690, .T. ) ;
#42855=EDGE_CURVE ( 'NONE', #8476, #81572, #15739, .T. ) ;
#42856=DIRECTION ( 'NONE',  ( 0.000000000000000000, 0.000000000000000000, -1.000000000000000000 ) ) ;
#42857=CARTESIAN_POINT ( 'NONE',  ( -12.89999999999999147, 2.500000000000000000, 3.637306695894644726 ) ) ;
#42858=DIRECTION ( 'NONE',  ( -0.000000000000000000, -1.000000000000000000, -0.000000000000000000 ) ) ;
#42859=DIRECTION ( 'NONE',  ( -0.000000000000000000, 1.000000000000000000, -0.000000000000000000 ) ) ;
#42860=DIRECTION ( 'NONE',  ( 0.000000000000000000, 1.000000000000000000, 0.000000000000000000 ) ) ;
#42861=CARTESIAN_POINT ( 'NONE',  ( 11.24999999999990585, 12.50000000000000000, -5.737276932171712751 ) ) ;
#42862=DIRECTION ( 'NONE',  ( 0.000000000000000000, 0.000000000000000000, -1.000000000000000000 ) ) ;
#42863=CIRCLE ( 'NONE', #51267, 0.06509327318403745899 ) ;
#42864=ORIENTED_EDGE ( 'NONE', *, *, #90518, .F. ) ;
#42865=VERTEX_POINT ( 'NONE', #83404 ) ;
#42866=ORIENTED_EDGE ( 'NONE', *, *, #102191, .F. ) ;
#42867=ORIENTED_EDGE ( 'NONE', *, *, #98933, .F. ) ;
#42868=DIRECTION ( 'NONE',  ( 0.000000000000000000, 1.000000000000000000, 0.000000000000000000 ) ) ;
#42869=PLANE ( 'NONE',  #43599 ) ;
#42870=CARTESIAN_POINT ( 'NONE',  ( 11.84999999999990727, 12.50000000000000000, 6.776507416713035248 ) ) ;
#42871=ORIENTED_EDGE ( 'NONE', *, *, #123535, .T. ) ;
#42872=FACE_BOUND ( 'NONE', #5715, .T. ) ;
#42873=ADVANCED_FACE ( 'NONE', ( #24473 ), #1596, .T. ) ;
#42875=FACE_OUTER_BOUND ( 'NONE', #36657, .T. ) ;
#42876=CIRCLE ( 'NONE', #93023, 0.09999999999999982514 ) ;
#42877=DIRECTION ( 'NONE',  ( 0.000000000000000000, 1.000000000000000000, 0.000000000000000000 ) ) ;
#42878=DIRECTION ( 'NONE',  ( 0.000000000000000000, 0.000000000000000000, -1.000000000000000000 ) ) ;
#42879=CONICAL_SURFACE ( 'NONE', #97219, 0.1000000000000002554, 0.003490658503988666988 ) ;
#42880=CARTESIAN_POINT ( 'NONE',  ( -7.950000000000016165, 12.50000000000000000, -6.560283801567334372 ) ) ;
#42881=CARTESIAN_POINT ( 'NONE',  ( 10.19999999999991402, 2.500000000000000000, 0.2464101615137735679 ) ) ;
#42882=CARTESIAN_POINT ( 'NONE',  ( -12.49999999999999289, 2.500000000000000000, 5.122947341949749323 ) ) ;
#42883=CARTESIAN_POINT ( 'NONE',  ( 14.14999999999989377, 12.50000000000000000, -2.857883832488653741 ) ) ;
#42884=EDGE_LOOP ( 'NONE', ( #47182, #93711, #23614, #92927 ) ) ;
#42885=CIRCLE ( 'NONE', #122290, 0.1000000000000002554 ) ;
#42886=EDGE_LOOP ( 'NONE', ( #46376, #84472 ) ) ;
#42888=AXIS2_PLACEMENT_3D ( 'NONE', #114168, #15939, #46712 ) ;
#42889=ADVANCED_FACE ( 'NONE', ( #62481 ), #61750, .T. ) ;
#42890=ORIENTED_EDGE ( 'NONE', *, *, #121513, .F. ) ;
#42891=ORIENTED_EDGE ( 'NONE', *, *, #109572, .T. ) ;
#42892=ORIENTED_EDGE ( 'NONE', *, *, #65718, .F. ) ;
#42893=DIRECTION ( 'NONE',  ( 0.000000000000000000, 0.000000000000000000, 1.000000000000000000 ) ) ;
#42894=ORIENTED_EDGE ( 'NONE', *, *, #92393, .T. ) ;
#42896=DIRECTION ( 'NONE',  ( -4.274815082592931898E-19, -0.9999939076577903929, -0.003490651415223739937 ) ) ;
#42897=DIRECTION ( 'NONE',  ( 0.000000000000000000, 0.000000000000000000, -1.000000000000000000 ) ) ;
#42899=EDGE_CURVE ( 'NONE', #44047, #4826, #26226, .T. ) ;
#42900=CONICAL_SURFACE ( 'NONE', #105569, 0.1000000000000002554, 0.003490658503988666988 ) ;
#42901=ORIENTED_EDGE ( 'NONE', *, *, #32445, .F. ) ;
#42902=CARTESIAN_POINT ( 'NONE',  ( 5.399999999999932854, 2.500000000000000000, 3.637306695894644726 ) ) ;
#42903=EDGE_LOOP ( 'NONE', ( #108372, #70128, #110442, #68691 ) ) ;
#42904=AXIS2_PLACEMENT_3D ( 'NONE', #22810, #33895, #52253 ) ;
#42905=VERTEX_POINT ( 'NONE', #23834 ) ;
#42906=DIRECTION ( 'NONE',  ( 0.000000000000000000, -0.9999939076577903929, 0.003490651415223739937 ) ) ;
#42907=AXIS2_PLACEMENT_3D ( 'NONE', #99760, #120040, #47436 ) ;
#42908=CONICAL_SURFACE ( 'NONE', #111844, 0.1000000000000002554, 0.003490658503988666988 ) ;
#42909=CARTESIAN_POINT ( 'NONE',  ( -2.050000000000032685, 12.50000000000000000, -6.495190528383302464 ) ) ;
#42910=ADVANCED_FACE ( 'NONE', ( #44104 ), #113958, .T. ) ;
#42911=ORIENTED_EDGE ( 'NONE', *, *, #60821, .T. ) ;
#42912=ORIENTED_EDGE ( 'NONE', *, *, #41878, .F. ) ;
#42913=CARTESIAN_POINT ( 'NONE',  ( 9.149999999999915090, 12.50000000000000000, 6.495190528383297135 ) ) ;
#42914=VECTOR ( 'NONE', #78330, 1000.000000000000000 ) ;
#42915=AXIS2_PLACEMENT_3D ( 'NONE', #92935, #83114, #63469 ) ;
#42916=VECTOR ( 'NONE', #20852, 1000.000000000000000 ) ;
#42917=LINE ( 'NONE', #52074, #99752 ) ;
#42918=DIRECTION ( 'NONE',  ( -0.000000000000000000, -1.000000000000000000, -0.000000000000000000 ) ) ;
#42919=DIRECTION ( 'NONE',  ( 0.000000000000000000, -0.9999939076577903929, 0.003490651415223739937 ) ) ;
#42920=CIRCLE ( 'NONE', #30298, 0.06509327318403745899 ) ;
#42921=DIRECTION ( 'NONE',  ( 0.000000000000000000, 1.000000000000000000, 0.000000000000000000 ) ) ;
#42922=ORIENTED_EDGE ( 'NONE', *, *, #128334, .T. ) ;
#42923=CARTESIAN_POINT ( 'NONE',  ( 2.299999999999949640, 12.50000000000000000, -0.3464101615137782364 ) ) ;
#42924=AXIS2_PLACEMENT_3D ( 'NONE', #32481, #71730, #20701 ) ;
#42925=VECTOR ( 'NONE', #984, 1000.000000000000000 ) ;
#42926=ORIENTED_EDGE ( 'NONE', *, *, #21934, .F. ) ;
#42927=CARTESIAN_POINT ( 'NONE',  ( 87.50000000000001421, 6.099025433955699960, -4.412011999987998756 ) ) ;
#42928=ADVANCED_FACE ( 'NONE', ( #82767 ), #24081, .T. ) ;
#42929=ORIENTED_EDGE ( 'NONE', *, *, #382, .F. ) ;
#42930=DIRECTION ( 'NONE',  ( 0.000000000000000000, 0.000000000000000000, -1.000000000000000000 ) ) ;
#42931=CARTESIAN_POINT ( 'NONE',  ( -9.600000000000008527, 2.500000000000000000, -5.022947341949749678 ) ) ;
#42932=AXIS2_PLACEMENT_3D ( 'NONE', #49223, #106813, #129075 ) ;
#42933=CARTESIAN_POINT ( 'NONE',  ( -8.749999999999976907, 2.500000000000000000, -6.395190528383296602 ) ) ;
#42934=CARTESIAN_POINT ( 'NONE',  ( -10.65000000000000213, 2.500000000000000000, 6.841600689897072485 ) ) ;
#42935=ORIENTED_EDGE ( 'NONE', *, *, #91105, .F. ) ;
#42936=EDGE_CURVE ( 'NONE', #39885, #95740, #92564, .T. ) ;
#42937=FACE_OUTER_BOUND ( 'NONE', #127659, .T. ) ;
#42938=DIRECTION ( 'NONE',  ( -0.000000000000000000, -1.000000000000000000, -0.000000000000000000 ) ) ;
#42939=ORIENTED_EDGE ( 'NONE', *, *, #109686, .F. ) ;
#42941=EDGE_CURVE ( 'NONE', #75000, #22575, #95179, .T. ) ;
#42942=EDGE_CURVE ( 'NONE', #66987, #5464, #71636, .T. ) ;
#42943=ORIENTED_EDGE ( 'NONE', *, *, #11788, .F. ) ;
#42944=CARTESIAN_POINT ( 'NONE',  ( 17.50000000000000000, -0.9166666666666695162, 3.432456362931491700 ) ) ;
#42945=DIRECTION ( 'NONE',  ( 0.000000000000000000, 0.000000000000000000, 1.000000000000000000 ) ) ;
#42946=ADVANCED_FACE ( 'NONE', ( #112213 ), #74251, .T. ) ;
#42948=ADVANCED_FACE ( 'NONE', ( #93223 ), #122471, .T. ) ;
#42950=CARTESIAN_POINT ( 'NONE',  ( -5.000000000000023093, 2.500000000000000000, 0.6928203230275494784 ) ) ;
#42951=CARTESIAN_POINT ( 'NONE',  ( -2.300000000000033573, 2.500000000000000000, -3.983716857408426293 ) ) ;
#42952=DIRECTION ( 'NONE',  ( 0.000000000000000000, 0.000000000000000000, 1.000000000000000000 ) ) ;
#42953=FACE_OUTER_BOUND ( 'NONE', #59571, .T. ) ;
#42954=ADVANCED_FACE ( 'NONE', ( #91925 ), #63874, .T. ) ;
#42955=EDGE_CURVE ( 'NONE', #76244, #3965, #82766, .T. ) ;
#42956=AXIS2_PLACEMENT_3D ( 'NONE', #83887, #85817, #125733 ) ;
#42957=EDGE_CURVE ( 'NONE', #89603, #59130, #103688, .T. ) ;
#42958=VECTOR ( 'NONE', #112861, 1000.000000000000000 ) ;
#42959=EDGE_CURVE ( 'NONE', #128096, #34323, #32607, .T. ) ;
#42960=DIRECTION ( 'NONE',  ( -4.274815082592931898E-19, -0.9999939076577903929, -0.003490651415223739937 ) ) ;
#42961=EDGE_CURVE ( 'NONE', #106163, #27262, #7426, .T. ) ;
#42962=ORIENTED_EDGE ( 'NONE', *, *, #125825, .F. ) ;
#42963=CARTESIAN_POINT ( 'NONE',  ( 15.19999999999989271, 12.50000000000000000, -0.4115034346978157509 ) ) ;
#42964=CARTESIAN_POINT ( 'NONE',  ( -0.4000000000000404898, 12.50000000000000000, 4.957854068765711553 ) ) ;
#42965=PLANE ( 'NONE',  #56918 ) ;
#42966=PLANE ( 'NONE',  #4116 ) ;
#42967=EDGE_CURVE ( 'NONE', #112113, #30658, #68070, .T. ) ;
#42968=ORIENTED_EDGE ( 'NONE', *, *, #2932, .F. ) ;
#42969=CARTESIAN_POINT ( 'NONE',  ( -2.300000000000032685, 12.50000000000000000, -0.3464101615137783474 ) ) ;
#42970=VECTOR ( 'NONE', #10575, 1000.000000000000000 ) ;
#42971=AXIS2_PLACEMENT_3D ( 'NONE', #24657, #94038, #105792 ) ;
#42972=DIRECTION ( 'NONE',  ( 0.000000000000000000, -0.000000000000000000, 1.000000000000000000 ) ) ;
#42973=DIRECTION ( 'NONE',  ( 0.000000000000000000, 0.000000000000000000, 1.000000000000000000 ) ) ;
#42974=EDGE_LOOP ( 'NONE', ( #99479, #40980, #32622, #94285 ) ) ;
#42975=ORIENTED_EDGE ( 'NONE', *, *, #125098, .T. ) ;
#42976=CARTESIAN_POINT ( 'NONE',  ( 9.149999999999920419, 2.500000000000000000, -5.802370205355749988 ) ) ;
#42977=AXIS2_PLACEMENT_3D ( 'NONE', #116213, #77575, #84825 ) ;
#42978=CIRCLE ( 'NONE', #49232, 0.09999999999999982514 ) ;
#42979=ORIENTED_EDGE ( 'NONE', *, *, #67633, .T. ) ;
#42980=VERTEX_POINT ( 'NONE', #33650 ) ;
#42981=DIRECTION ( 'NONE',  ( 0.000000000000000000, -0.9999939076577903929, 0.003490651415223739937 ) ) ;
#42982=CARTESIAN_POINT ( 'NONE',  ( -3.150000000000030109, 12.50000000000000000, -2.511473670974877948 ) ) ;
#42983=DIRECTION ( 'NONE',  ( 0.000000000000000000, 0.000000000000000000, 1.000000000000000000 ) ) ;
#42984=CARTESIAN_POINT ( 'NONE',  ( 3.549999999999943867, 12.50000000000000000, -1.818653347947326138 ) ) ;
#42985=ORIENTED_EDGE ( 'NONE', *, *, #78799, .F. ) ;
#42986=AXIS2_PLACEMENT_3D ( 'NONE', #71855, #12266, #22127 ) ;
#42987=FACE_OUTER_BOUND ( 'NONE', #115780, .T. ) ;
#42988=DIRECTION ( 'NONE',  ( 0.000000000000000000, 0.000000000000000000, -1.000000000000000000 ) ) ;
#42989=EDGE_LOOP ( 'NONE', ( #50452, #8572, #78959, #57376 ) ) ;
#42990=CARTESIAN_POINT ( 'NONE',  ( 16.55874544816223448, 0.4845305829267578801, 6.091953208799004926 ) ) ;
#42991=DIRECTION ( 'NONE',  ( 0.000000000000000000, 0.000000000000000000, 1.000000000000000000 ) ) ;
#42992=AXIS2_PLACEMENT_3D ( 'NONE', #107923, #86993, #9078 ) ;
#42993=ORIENTED_EDGE ( 'NONE', *, *, #62769, .F. ) ;
#42994=EDGE_CURVE ( 'NONE', #118519, #9515, #120316, .T. ) ;
#42995=AXIS2_PLACEMENT_3D ( 'NONE', #27078, #48016, #48652 ) ;
#42996=VERTEX_POINT ( 'NONE', #34310 ) ;
#42997=CIRCLE ( 'NONE', #61855, 0.1000000000000002554 ) ;
#42998=ADVANCED_FACE ( 'NONE', ( #55228 ), #36701, .T. ) ;
#42999=ORIENTED_EDGE ( 'NONE', *, *, #71949, .F. ) ;
#43000=ORIENTED_EDGE ( 'NONE', *, *, #35785, .F. ) ;
#43001=CARTESIAN_POINT ( 'NONE',  ( 11.04999999999990834, 2.500000000000000000, 1.818653347947321475 ) ) ;
#43002=CARTESIAN_POINT ( 'NONE',  ( 15.83209681635555377, 2.499999999999999556, 5.404881881984140435 ) ) ;
#43003=CARTESIAN_POINT ( 'NONE',  ( 8.149999999999923972, 12.50000000000000000, 2.511473670974873507 ) ) ;
#43004=FACE_BOUND ( 'NONE', #99881, .T. ) ;
#43005=ORIENTED_EDGE ( 'NONE', *, *, #985, .F. ) ;
#43007=CARTESIAN_POINT ( 'NONE',  ( -9.800000000000006040, 2.500000000000000000, 0.4464101615137735513 ) ) ;
#43008=CARTESIAN_POINT ( 'NONE',  ( 10.64999999999991331, 2.500000000000000000, 6.148780366869520897 ) ) ;
#43009=VECTOR ( 'NONE', #87158, 1000.000000000000000 ) ;
#43010=EDGE_CURVE ( 'NONE', #13366, #26403, #24165, .T. ) ;
#43011=CARTESIAN_POINT ( 'NONE',  ( -0.6000000000000388356, 2.500000000000000000, 4.083716857408421497 ) ) ;
#43012=VECTOR ( 'NONE', #63219, 1000.000000000000000 ) ;
#43013=LINE ( 'NONE', #90787, #96928 ) ;
#43014=DIRECTION ( 'NONE',  ( 0.000000000000000000, 0.000000000000000000, -1.000000000000000000 ) ) ;
#43015=AXIS2_PLACEMENT_3D ( 'NONE', #16012, #97806, #127285 ) ;
#43016=AXIS2_PLACEMENT_3D ( 'NONE', #106273, #56520, #47359 ) ;
#43017=DIRECTION ( 'NONE',  ( -0.000000000000000000, 1.000000000000000000, -0.000000000000000000 ) ) ;
#43018=AXIS2_PLACEMENT_3D ( 'NONE', #8717, #66370, #118046 ) ;
#43019=ORIENTED_EDGE ( 'NONE', *, *, #49282, .F. ) ;
#43020=ORIENTED_EDGE ( 'NONE', *, *, #119132, .T. ) ;
#43021=VERTEX_POINT ( 'NONE', #46689 ) ;
#43022=EDGE_LOOP ( 'NONE', ( #105006, #10359, #10498, #32605 ) ) ;
#43023=AXIS2_PLACEMENT_3D ( 'NONE', #95573, #3321, #93000 ) ;
#43024=VERTEX_POINT ( 'NONE', #4808 ) ;
#43025=DIRECTION ( 'NONE',  ( 0.000000000000000000, 0.000000000000000000, 1.000000000000000000 ) ) ;
#43026=DIRECTION ( 'NONE',  ( 0.000000000000000000, -0.9999939076577903929, 0.003490651415223739937 ) ) ;
#43027=ORIENTED_EDGE ( 'NONE', *, *, #114636, .F. ) ;
#43028=FACE_BOUND ( 'NONE', #71927, .T. ) ;
#43029=PLANE ( 'NONE',  #110467 ) ;
#43030=EDGE_LOOP ( 'NONE', ( #53489, #7251, #5658, #26336 ) ) ;
#43031=CARTESIAN_POINT ( 'NONE',  ( 7.099999999999927702, 12.50000000000000000, 5.022947341949748790 ) ) ;
#43032=DIRECTION ( 'NONE',  ( -0.000000000000000000, -1.000000000000000000, -0.000000000000000000 ) ) ;
#43033=CARTESIAN_POINT ( 'NONE',  ( 4.799999999999935874, 12.50000000000000000, 0.3464101615137735735 ) ) ;
#43034=CIRCLE ( 'NONE', #116153, 0.09999999999999999167 ) ;
#43035=ORIENTED_EDGE ( 'NONE', *, *, #34649, .T. ) ;
#43036=DIRECTION ( 'NONE',  ( -0.000000000000000000, -1.000000000000000000, -0.000000000000000000 ) ) ;
#43037=EDGE_CURVE ( 'NONE', #23590, #15508, #9593, .T. ) ;
#43038=ORIENTED_EDGE ( 'NONE', *, *, #68365, .T. ) ;
#43039=ORIENTED_EDGE ( 'NONE', *, *, #118188, .F. ) ;
#43040=VERTEX_POINT ( 'NONE', #27673 ) ;
#43041=CARTESIAN_POINT ( 'NONE',  ( 11.44999999999990692, 12.50000000000000000, -6.841600689897078702 ) ) ;
#43042=CARTESIAN_POINT ( 'NONE',  ( 8.749999999999918288, 12.50000000000000000, 7.188010851410848723 ) ) ;
#43043=CIRCLE ( 'NONE', #76468, 0.06509327318403745899 ) ;
#43044=CARTESIAN_POINT ( 'NONE',  ( -6.450000000000016165, 12.50000000000000000, 2.511473670974873507 ) ) ;
#43045=EDGE_LOOP ( 'NONE', ( #9479, #59827, #89140, #60459 ) ) ;
#43046=CARTESIAN_POINT ( 'NONE',  ( -12.09999999999999432, 2.500000000000000000, 3.637306695894644726 ) ) ;
#43047=AXIS2_PLACEMENT_3D ( 'NONE', #15922, #46694, #86605 ) ;
#43048=DIRECTION ( 'NONE',  ( 0.000000000000000000, 0.000000000000000000, 1.000000000000000000 ) ) ;
#43049=AXIS2_PLACEMENT_3D ( 'NONE', #60386, #100916, #30276 ) ;
#43050=DIRECTION ( 'NONE',  ( 0.000000000000000000, 0.000000000000000000, 1.000000000000000000 ) ) ;
#43052=VERTEX_POINT ( 'NONE', #26416 ) ;
#43053=EDGE_CURVE ( 'NONE', #69984, #84331, #128750, .T. ) ;
#43054=DIRECTION ( 'NONE',  ( 0.000000000000000000, -0.000000000000000000, 1.000000000000000000 ) ) ;
#43055=ADVANCED_FACE ( 'NONE', ( #36235 ), #104319, .T. ) ;
#43056=ORIENTED_EDGE ( 'NONE', *, *, #128983, .T. ) ;
#43057=CARTESIAN_POINT ( 'NONE',  ( 6.249999999999928946, 2.500000000000000000, 2.957883832488649389 ) ) ;
#43058=AXIS2_PLACEMENT_3D ( 'NONE', #11068, #9153, #79825 ) ;
#43059=ORIENTED_EDGE ( 'NONE', *, *, #72640, .T. ) ;
#43060=AXIS2_PLACEMENT_3D ( 'NONE', #37702, #70868, #57336 ) ;
#43061=ORIENTED_EDGE ( 'NONE', *, *, #125890, .T. ) ;
#43062=FACE_OUTER_BOUND ( 'NONE', #114662, .T. ) ;
#43063=DIRECTION ( 'NONE',  ( -0.000000000000000000, 1.000000000000000000, -0.000000000000000000 ) ) ;
#43064=DIRECTION ( 'NONE',  ( -0.000000000000000000, -1.000000000000000000, -0.000000000000000000 ) ) ;
#43065=FACE_OUTER_BOUND ( 'NONE', #121088, .T. ) ;
#43066=ADVANCED_FACE ( 'NONE', ( #84676 ), #105732, .T. ) ;
#43067=DIRECTION ( 'NONE',  ( 0.000000000000000000, 0.000000000000000000, 1.000000000000000000 ) ) ;
#43068=VERTEX_POINT ( 'NONE', #6099 ) ;
#43069=ORIENTED_EDGE ( 'NONE', *, *, #79145, .T. ) ;
#43070=DIRECTION ( 'NONE',  ( 0.000000000000000000, 0.000000000000000000, -1.000000000000000000 ) ) ;
#43071=VECTOR ( 'NONE', #6727, 1000.000000000000000 ) ;
#43072=VECTOR ( 'NONE', #98225, 1000.000000000000000 ) ;
#43074=CARTESIAN_POINT ( 'NONE',  ( 10.84999999999991260, 12.50000000000000000, 5.867463478539781896 ) ) ;
#43075=ORIENTED_EDGE ( 'NONE', *, *, #80019, .T. ) ;
#43076=ORIENTED_EDGE ( 'NONE', *, *, #17277, .F. ) ;
#43077=DIRECTION ( 'NONE',  ( 0.000000000000000000, 1.000000000000000000, 0.000000000000000000 ) ) ;
#43078=VERTEX_POINT ( 'NONE', #55856 ) ;
#43079=DIRECTION ( 'NONE',  ( 0.000000000000000000, 0.000000000000000000, -1.000000000000000000 ) ) ;
#43080=FACE_OUTER_BOUND ( 'NONE', #31601, .T. ) ;
#43081=FACE_OUTER_BOUND ( 'NONE', #101672, .T. ) ;
#43082=ORIENTED_EDGE ( 'NONE', *, *, #48257, .T. ) ;
#43083=CARTESIAN_POINT ( 'NONE',  ( -2.500000000000031086, 12.50000000000000000, 3.637306695894644726 ) ) ;
#43084=CARTESIAN_POINT ( 'NONE',  ( 14.14999999999989200, 2.500000000000000000, -2.065063509461102065 ) ) ;
#43085=DIRECTION ( 'NONE',  ( -0.000000000000000000, 1.000000000000000000, -0.000000000000000000 ) ) ;
#43086=DIRECTION ( 'NONE',  ( -0.000000000000000000, -1.000000000000000000, -0.000000000000000000 ) ) ;
#43087=CARTESIAN_POINT ( 'NONE',  ( 7.299999999999926104, 12.50000000000000000, -4.048810130592463530 ) ) ;
#43088=ORIENTED_EDGE ( 'NONE', *, *, #66979, .T. ) ;
#43090=FACE_OUTER_BOUND ( 'NONE', #91574, .T. ) ;
#43091=AXIS2_PLACEMENT_3D ( 'NONE', #9922, #99604, #37467 ) ;
#43092=CARTESIAN_POINT ( 'NONE',  ( 26.61818291006423109, -2.722754637273441691, 4.358315985292433581 ) ) ;
#43093=ORIENTED_EDGE ( 'NONE', *, *, #65788, .T. ) ;
#43094=EDGE_LOOP ( 'NONE', ( #87186, #27036 ) ) ;
#43095=EDGE_CURVE ( 'NONE', #87886, #70557, #66018, .T. ) ;
#43097=DIRECTION ( 'NONE',  ( 0.000000000000000000, 0.000000000000000000, 1.000000000000000000 ) ) ;
#43098=CARTESIAN_POINT ( 'NONE',  ( -3.100000000000028511, 2.500000000000000000, 0.4464101615137736623 ) ) ;
#43099=EDGE_CURVE ( 'NONE', #45964, #68456, #55562, .T. ) ;
#43100=CARTESIAN_POINT ( 'NONE',  ( -9.150000000000009237, 2.500000000000000000, -2.957883832488653830 ) ) ;
#43101=DIRECTION ( 'NONE',  ( 0.000000000000000000, 0.000000000000000000, -1.000000000000000000 ) ) ;
#43102=LINE ( 'NONE', #83648, #34581 ) ;
#43103=CARTESIAN_POINT ( 'NONE',  ( -2.950000000000029932, 2.500000000000000000, 2.165063509461097713 ) ) ;
#43104=CARTESIAN_POINT ( 'NONE',  ( -9.150000000000009237, 2.500000000000000000, -6.495190528383297135 ) ) ;
#43105=CARTESIAN_POINT ( 'NONE',  ( -11.64999999999999858, 2.500000000000000000, -5.902370205355746968 ) ) ;
#43106=EDGE_CURVE ( 'NONE', #90933, #77506, #74865, .T. ) ;
#43107=EDGE_CURVE ( 'NONE', #39770, #122938, #22135, .T. ) ;
#43108=EDGE_CURVE ( 'NONE', #45836, #67411, #25108, .T. ) ;
#43109=CARTESIAN_POINT ( 'NONE',  ( -2.500000000000032419, 2.500000000000000000, -3.537306695894649966 ) ) ;
#43110=ORIENTED_EDGE ( 'NONE', *, *, #81357, .F. ) ;
#43111=VERTEX_POINT ( 'NONE', #126546 ) ;
#43112=CIRCLE ( 'NONE', #84835, 0.06509327318403745899 ) ;
#43113=EDGE_CURVE ( 'NONE', #124524, #67119, #95272, .T. ) ;
#43114=EDGE_LOOP ( 'NONE', ( #111223, #14874 ) ) ;
#43115=CIRCLE ( 'NONE', #55604, 0.06509327318403745899 ) ;
#43116=EDGE_LOOP ( 'NONE', ( #2976, #45642 ) ) ;
#43117=CARTESIAN_POINT ( 'NONE',  ( -10.45000000000000107, 12.50000000000000000, 2.230156782645134950 ) ) ;
#43118=CARTESIAN_POINT ( 'NONE',  ( 5.649999999999934630, 12.50000000000000000, -2.511473670974877948 ) ) ;
#43119=EDGE_CURVE ( 'NONE', #30275, #24551, #56495, .T. ) ;
#43120=ORIENTED_EDGE ( 'NONE', *, *, #968, .T. ) ;
#43121=DIRECTION ( 'NONE',  ( 0.000000000000000000, 0.000000000000000000, -1.000000000000000000 ) ) ;
#43122=LINE ( 'NONE', #83035, #13538 ) ;
#43123=CARTESIAN_POINT ( 'NONE',  ( -3.100000000000028511, 12.50000000000000000, 0.3464101615137736845 ) ) ;
#43124=VERTEX_POINT ( 'NONE', #27052 ) ;
#43125=FACE_OUTER_BOUND ( 'NONE', #115369, .T. ) ;
#43126=DIRECTION ( 'NONE',  ( -0.000000000000000000, -1.000000000000000000, -0.000000000000000000 ) ) ;
#43127=VERTEX_POINT ( 'NONE', #106879 ) ;
#43128=AXIS2_PLACEMENT_3D ( 'NONE', #47749, #27437, #108591 ) ;
#43129=ORIENTED_EDGE ( 'NONE', *, *, #76014, .T. ) ;
#43130=EDGE_LOOP ( 'NONE', ( #16569, #113783 ) ) ;
#43131=EDGE_LOOP ( 'NONE', ( #13304, #80860, #117388, #125603 ) ) ;
#43132=CARTESIAN_POINT ( 'NONE',  ( 1.249999999999952482, 12.50000000000000000, -5.802370205355749988 ) ) ;
#43133=AXIS2_PLACEMENT_3D ( 'NONE', #107245, #126248, #47051 ) ;
#43134=LINE ( 'NONE', #92865, #25830 ) ;
#43135=DIRECTION ( 'NONE',  ( 0.000000000000000000, 0.000000000000000000, 1.000000000000000000 ) ) ;
#43136=AXIS2_PLACEMENT_3D ( 'NONE', #79385, #47346, #87245 ) ;
#43137=CARTESIAN_POINT ( 'NONE',  ( -4.350000000000023626, 2.500000000000000000, -2.411473670974877859 ) ) ;
#43138=ORIENTED_EDGE ( 'NONE', *, *, #95561, .F. ) ;
#43139=AXIS2_PLACEMENT_3D ( 'NONE', #28829, #99503, #79843 ) ;
#43140=DIRECTION ( 'NONE',  ( 0.000000000000000000, 1.000000000000000000, 0.000000000000000000 ) ) ;
#43141=VERTEX_POINT ( 'NONE', #15264 ) ;
#43142=PLANE ( 'NONE',  #18293 ) ;
#43143=CARTESIAN_POINT ( 'NONE',  ( 7.173569985889933776, -2.500000000000000000, -8.713264184204838614 ) ) ;
#43144=PLANE ( 'NONE',  #60933 ) ;
#43145=DIRECTION ( 'NONE',  ( -0.000000000000000000, -1.000000000000000000, -0.000000000000000000 ) ) ;
#43146=AXIS2_PLACEMENT_3D ( 'NONE', #104614, #76460, #126198 ) ;
#43147=VERTEX_POINT ( 'NONE', #45412 ) ;
#43148=EDGE_CURVE ( 'NONE', #112146, #45854, #7390, .T. ) ;
#43149=VECTOR ( 'NONE', #69926, 1000.000000000000000 ) ;
#43150=AXIS2_PLACEMENT_3D ( 'NONE', #5332, #47208, #24983 ) ;
#43151=ORIENTED_EDGE ( 'NONE', *, *, #29533, .T. ) ;
#43152=ORIENTED_EDGE ( 'NONE', *, *, #118049, .T. ) ;
#43153=DIRECTION ( 'NONE',  ( -0.000000000000000000, -1.000000000000000000, -0.000000000000000000 ) ) ;
#43154=CARTESIAN_POINT ( 'NONE',  ( -3.642919299551294898E-14, 2.500000000000000000, 0.6928203230275518099 ) ) ;
#43155=DIRECTION ( 'NONE',  ( -0.000000000000000000, 1.000000000000000000, -0.000000000000000000 ) ) ;
#43156=FACE_BOUND ( 'NONE', #85104, .T. ) ;
#43157=CARTESIAN_POINT ( 'NONE',  ( -5.800000000000018474, 2.500000000000000000, 4.330127018922196314 ) ) ;
#43158=DIRECTION ( 'NONE',  ( 0.000000000000000000, 0.000000000000000000, -1.000000000000000000 ) ) ;
#43159=CARTESIAN_POINT ( 'NONE',  ( 7.499999999999927169, 12.50000000000000000, -5.022947341949754119 ) ) ;
#43160=EDGE_CURVE ( 'NONE', #88434, #58364, #59795, .T. ) ;
#43161=CARTESIAN_POINT ( 'NONE',  ( 9.399999999999918643, 12.50000000000000000, 0.3464101615137736845 ) ) ;
#43163=CARTESIAN_POINT ( 'NONE',  ( 1.899999999999949507, 2.500000000000000000, 4.083716857408421497 ) ) ;
#43164=ORIENTED_EDGE ( 'NONE', *, *, #108351, .T. ) ;
#43165=CARTESIAN_POINT ( 'NONE',  ( -6.900000000000015454, 12.50000000000000000, 4.048810130592458201 ) ) ;
#43166=ORIENTED_EDGE ( 'NONE', *, *, #9284, .T. ) ;
#43168=CARTESIAN_POINT ( 'NONE',  ( -0.4000000000000396572, 12.50000000000000000, 3.572213422710607489 ) ) ;
#43169=DIRECTION ( 'NONE',  ( 0.000000000000000000, 0.000000000000000000, -1.000000000000000000 ) ) ;
#43170=FACE_BOUND ( 'NONE', #29278, .T. ) ;
#43171=CARTESIAN_POINT ( 'NONE',  ( -11.64999999999999680, 2.500000000000000000, -7.188010851410850499 ) ) ;
#43172=CIRCLE ( 'NONE', #30563, 0.1000000000000002554 ) ;
#43173=AXIS2_PLACEMENT_3D ( 'NONE', #26834, #58872, #58242 ) ;
#43174=EDGE_LOOP ( 'NONE', ( #29167, #60920, #46364, #119367 ) ) ;
#43175=CARTESIAN_POINT ( 'NONE',  ( 87.49999999944498086, 3.974992050012154277, 6.359987280019447020 ) ) ;
#43176=FACE_OUTER_BOUND ( 'NONE', #118483, .T. ) ;
#43177=ORIENTED_EDGE ( 'NONE', *, *, #109226, .T. ) ;
#43178=CARTESIAN_POINT ( 'NONE',  ( -2.700000000000031264, 12.50000000000000000, 4.676537180435972552 ) ) ;
#43179=DIRECTION ( 'NONE',  ( 0.000000000000000000, 1.000000000000000000, 0.000000000000000000 ) ) ;
#43180=CONICAL_SURFACE ( 'NONE', #61947, 0.1000000000000002554, 0.003490658503988666988 ) ;
#43182=ADVANCED_FACE ( 'NONE', ( #109475 ), #38835, .T. ) ;
#43183=EDGE_LOOP ( 'NONE', ( #110829, #26599 ) ) ;
#43184=FACE_OUTER_BOUND ( 'NONE', #35819, .T. ) ;
#43185=DIRECTION ( 'NONE',  ( 0.000000000000000000, 0.000000000000000000, 1.000000000000000000 ) ) ;
#43186=AXIS2_PLACEMENT_3D ( 'NONE', #64813, #11841, #51785 ) ;
#43187=AXIS2_PLACEMENT_3D ( 'NONE', #13165, #60381, #93047 ) ;
#43188=ADVANCED_FACE ( 'NONE', ( #17862 ), #19132, .T. ) ;
#43189=ORIENTED_EDGE ( 'NONE', *, *, #29137, .T. ) ;
#43190=AXIS2_PLACEMENT_3D ( 'NONE', #74598, #4532, #52380 ) ;
#43191=DIRECTION ( 'NONE',  ( 0.000000000000000000, 0.000000000000000000, 1.000000000000000000 ) ) ;
#43192=DIRECTION ( 'NONE',  ( -0.000000000000000000, -1.000000000000000000, -0.000000000000000000 ) ) ;
#43193=CARTESIAN_POINT ( 'NONE',  ( 10.19999999999991225, 12.50000000000000000, -4.676537180435978769 ) ) ;
#43194=ORIENTED_EDGE ( 'NONE', *, *, #96816, .T. ) ;
#43195=EDGE_CURVE ( 'NONE', #47459, #20502, #26325, .T. ) ;
#43197=EDGE_CURVE ( 'NONE', #95641, #52044, #74335, .T. ) ;
#43198=EDGE_LOOP ( 'NONE', ( #103740, #65622 ) ) ;
#43199=DIRECTION ( 'NONE',  ( 0.000000000000000000, 0.000000000000000000, 1.000000000000000000 ) ) ;
#43200=DIRECTION ( 'NONE',  ( 0.000000000000000000, 0.000000000000000000, 1.000000000000000000 ) ) ;
#43201=EDGE_LOOP ( 'NONE', ( #16623, #61145 ) ) ;
#43202=EDGE_CURVE ( 'NONE', #3469, #100762, #116181, .T. ) ;
#43203=CARTESIAN_POINT ( 'NONE',  ( 12.69999999999990337, 12.50000000000000000, 3.983716857408420076 ) ) ;
#43204=CARTESIAN_POINT ( 'NONE',  ( -14.14999999999998614, 12.50000000000000000, 1.537336459617586915 ) ) ;
#43205=DIRECTION ( 'NONE',  ( 0.000000000000000000, 0.000000000000000000, 1.000000000000000000 ) ) ;
#43206=CARTESIAN_POINT ( 'NONE',  ( -4.150000000000028777, 2.500000000000000000, -5.902370205355750521 ) ) ;
#43207=EDGE_CURVE ( 'NONE', #127992, #110877, #101534, .T. ) ;
#43208=CONICAL_SURFACE ( 'NONE', #78708, 0.09999999999999982514, 0.003490658503988666988 ) ;
#43210=AXIS2_PLACEMENT_3D ( 'NONE', #116098, #44138, #116732 ) ;
#43211=VERTEX_POINT ( 'NONE', #40760 ) ;
#43212=VERTEX_POINT ( 'NONE', #88534 ) ;
#43213=DIRECTION ( 'NONE',  ( -0.000000000000000000, 1.000000000000000000, -0.000000000000000000 ) ) ;
#43214=VERTEX_POINT ( 'NONE', #68251 ) ;
#43215=VECTOR ( 'NONE', #94622, 1000.000000000000000 ) ;
#43217=ORIENTED_EDGE ( 'NONE', *, *, #26220, .F. ) ;
#43218=EDGE_LOOP ( 'NONE', ( #126246, #34996 ) ) ;
#43219=VERTEX_POINT ( 'NONE', #78750 ) ;
#43220=CARTESIAN_POINT ( 'NONE',  ( 1.049999999999954525, 12.50000000000000000, 1.818653347947321475 ) ) ;
#43221=VECTOR ( 'NONE', #118337, 1000.000000000000000 ) ;
#43222=CARTESIAN_POINT ( 'NONE',  ( 5.849999999999933031, 2.500000000000000000, 7.288010851410849256 ) ) ;
#43223=DIRECTION ( 'NONE',  ( 0.000000000000000000, 0.000000000000000000, 1.000000000000000000 ) ) ;
#43224=CONICAL_SURFACE ( 'NONE', #53585, 0.1000000000000000056, 0.003490658503988666988 ) ;
#43226=DIRECTION ( 'NONE',  ( 0.000000000000000000, -0.000000000000000000, 1.000000000000000000 ) ) ;
#43227=EDGE_CURVE ( 'NONE', #61297, #61474, #80670, .T. ) ;
#43228=DIRECTION ( 'NONE',  ( 0.000000000000000000, 0.000000000000000000, 1.000000000000000000 ) ) ;
#43229=CARTESIAN_POINT ( 'NONE',  ( -8.350000000000013856, 2.500000000000000000, -6.595190528383296780 ) ) ;
#43230=CARTESIAN_POINT ( 'NONE',  ( -12.04999999999999716, 2.500000000000000000, -6.595190528383298556 ) ) ;
#43231=DIRECTION ( 'NONE',  ( 0.000000000000000000, 0.000000000000000000, 1.000000000000000000 ) ) ;
#43232=AXIS2_PLACEMENT_3D ( 'NONE', #101476, #11791, #62207 ) ;
#43233=CARTESIAN_POINT ( 'NONE',  ( 7.899999999999921307, 2.500000000000000000, -2.385244779468109755E-15 ) ) ;
#43234=AXIS2_PLACEMENT_3D ( 'NONE', #86587, #117309, #18498 ) ;
#43235=ORIENTED_EDGE ( 'NONE', *, *, #121234, .T. ) ;
#43236=ADVANCED_FACE ( 'NONE', ( #80012 ), #19966, .T. ) ;
#43238=DIRECTION ( 'NONE',  ( -0.000000000000000000, 1.000000000000000000, -0.000000000000000000 ) ) ;
#43240=ORIENTED_EDGE ( 'NONE', *, *, #65832, .T. ) ;
#43241=CARTESIAN_POINT ( 'NONE',  ( 11.84999999999990727, 12.50000000000000000, -2.511473670974877948 ) ) ;
#43242=CARTESIAN_POINT ( 'NONE',  ( 5.849999999999933920, 12.50000000000000000, 6.495190528383297135 ) ) ;
#43243=DIRECTION ( 'NONE',  ( -0.000000000000000000, -1.000000000000000000, -0.000000000000000000 ) ) ;
#43244=EDGE_CURVE ( 'NONE', #35406, #81765, #5376, .T. ) ;
#43245=DIRECTION ( 'NONE',  ( 0.000000000000000000, 0.000000000000000000, 1.000000000000000000 ) ) ;
#43246=DIRECTION ( 'NONE',  ( 0.000000000000000000, 0.000000000000000000, 1.000000000000000000 ) ) ;
#43247=DIRECTION ( 'NONE',  ( 0.000000000000000000, 0.000000000000000000, 1.000000000000000000 ) ) ;
#43248=DIRECTION ( 'NONE',  ( 0.000000000000000000, -0.9999939076577903929, 0.003490651415223739937 ) ) ;
#43249=EDGE_LOOP ( 'NONE', ( #127345, #95620 ) ) ;
#43251=ADVANCED_FACE ( 'NONE', ( #23031 ), #102856, .T. ) ;
#43252=EDGE_CURVE ( 'NONE', #67756, #94856, #26897, .T. ) ;
#43253=DIRECTION ( 'NONE',  ( 0.000000000000000000, 0.000000000000000000, -1.000000000000000000 ) ) ;
#43254=ORIENTED_EDGE ( 'NONE', *, *, #42955, .T. ) ;
#43255=EDGE_LOOP ( 'NONE', ( #12538, #66709 ) ) ;
#43256=ADVANCED_FACE ( 'NONE', ( #96913 ), #101347, .T. ) ;
#43257=EDGE_LOOP ( 'NONE', ( #62934, #70235 ) ) ;
#43258=EDGE_LOOP ( 'NONE', ( #110164, #26468 ) ) ;
#43259=CARTESIAN_POINT ( 'NONE',  ( -2.500000000000030642, 12.50000000000000000, -0.6928203230275541413 ) ) ;
#43260=DIRECTION ( 'NONE',  ( -0.000000000000000000, -1.000000000000000000, -0.000000000000000000 ) ) ;
#43261=EDGE_CURVE ( 'NONE', #41869, #9888, #44908, .T. ) ;
#43262=EDGE_CURVE ( 'NONE', #63955, #110791, #99199, .T. ) ;
#43263=CIRCLE ( 'NONE', #9787, 0.06509327318403745899 ) ;
#43264=DIRECTION ( 'NONE',  ( 0.000000000000000000, 0.000000000000000000, 1.000000000000000000 ) ) ;
#43265=AXIS2_PLACEMENT_3D ( 'NONE', #11696, #32004, #81719 ) ;
#43266=DIRECTION ( 'NONE',  ( 0.000000000000000000, 1.000000000000000000, 0.000000000000000000 ) ) ;
#43267=CARTESIAN_POINT ( 'NONE',  ( -5.000000000000023093, 2.500000000000000000, 0.5928203230275495006 ) ) ;
#43269=DIRECTION ( 'NONE',  ( 0.000000000000000000, 0.000000000000000000, 1.000000000000000000 ) ) ;
#43270=CARTESIAN_POINT ( 'NONE',  ( -9.600000000000008527, 2.500000000000000000, -2.385244779468109755E-15 ) ) ;
#43271=DIRECTION ( 'NONE',  ( -0.000000000000000000, -1.000000000000000000, -0.000000000000000000 ) ) ;
#43272=VECTOR ( 'NONE', #83201, 1000.000000000000000 ) ;
#43273=AXIS2_PLACEMENT_3D ( 'NONE', #80013, #20457, #18514 ) ;
#43274=DIRECTION ( 'NONE',  ( 0.000000000000000000, 0.000000000000000000, 1.000000000000000000 ) ) ;
#43275=ORIENTED_EDGE ( 'NONE', *, *, #32851, .F. ) ;
#43276=EDGE_LOOP ( 'NONE', ( #122923, #124794, #18653, #27640 ) ) ;
#43277=ORIENTED_EDGE ( 'NONE', *, *, #22672, .T. ) ;
#43279=AXIS2_PLACEMENT_3D ( 'NONE', #69152, #35371, #118260 ) ;
#43280=LINE ( 'NONE', #33458, #17412 ) ;
#43281=CARTESIAN_POINT ( 'NONE',  ( -12.89999999999999147, 2.500000000000000000, -0.7928203230275501223 ) ) ;
#43282=AXIS2_PLACEMENT_3D ( 'NONE', #84033, #123962, #85959 ) ;
#43283=ORIENTED_EDGE ( 'NONE', *, *, #54776, .T. ) ;
#43284=DIRECTION ( 'NONE',  ( -4.274815082592931898E-19, -0.9999939076577903929, -0.003490651415223739937 ) ) ;
#43285=LINE ( 'NONE', #14429, #85052 ) ;
#43286=DIRECTION ( 'NONE',  ( 0.000000000000000000, 0.000000000000000000, 1.000000000000000000 ) ) ;
#43287=DIRECTION ( 'NONE',  ( 0.000000000000000000, -0.000000000000000000, 1.000000000000000000 ) ) ;
#43288=DIRECTION ( 'NONE',  ( 0.000000000000000000, 1.000000000000000000, 0.000000000000000000 ) ) ;
#43289=EDGE_CURVE ( 'NONE', #89858, #23588, #19774, .T. ) ;
#43290=VERTEX_POINT ( 'NONE', #56342 ) ;
#43291=ORIENTED_EDGE ( 'NONE', *, *, #110819, .F. ) ;
#43292=LINE ( 'NONE', #14438, #45977 ) ;
#43293=AXIS2_PLACEMENT_3D ( 'NONE', #43689, #32583, #83598 ) ;
#43294=CARTESIAN_POINT ( 'NONE',  ( 11.24999999999990941, 2.500000000000000000, -1.372243186433550033 ) ) ;
#43295=CIRCLE ( 'NONE', #116423, 0.1000000000000002554 ) ;
#43296=CARTESIAN_POINT ( 'NONE',  ( -5.000000000000022204, 12.50000000000000000, 3.702399969078682407 ) ) ;
#43298=DIRECTION ( 'NONE',  ( 0.000000000000000000, 0.000000000000000000, 1.000000000000000000 ) ) ;
#43299=EDGE_CURVE ( 'NONE', #58093, #7017, #65521, .T. ) ;
#43301=AXIS2_PLACEMENT_3D ( 'NONE', #122652, #91906, #33002 ) ;
#43302=ORIENTED_EDGE ( 'NONE', *, *, #24708, .T. ) ;
#43303=DIRECTION ( 'NONE',  ( 0.000000000000000000, -0.9999939076577903929, 0.003490651415223739937 ) ) ;
#43304=CARTESIAN_POINT ( 'NONE',  ( 9.999999999999912959, 2.500000000000000000, -4.922947341949753586 ) ) ;
#43305=AXIS2_PLACEMENT_3D ( 'NONE', #4990, #15456, #92754 ) ;
#43306=CARTESIAN_POINT ( 'NONE',  ( 16.88398418148221225, -2.500000000000000000, -4.430584152985939106 ) ) ;
#43307=DIRECTION ( 'NONE',  ( 0.000000000000000000, -0.9999939076577903929, 0.003490651415223739937 ) ) ;
#43308=DIRECTION ( 'NONE',  ( 0.000000000000000000, 0.000000000000000000, -1.000000000000000000 ) ) ;
#43309=ORIENTED_EDGE ( 'NONE', *, *, #38796, .F. ) ;
#43310=FACE_OUTER_BOUND ( 'NONE', #105539, .T. ) ;
#43311=CIRCLE ( 'NONE', #37040, 0.06509327318403745899 ) ;
#43312=CARTESIAN_POINT ( 'NONE',  ( 4.349999999999941025, 2.500000000000000000, -1.718653347947326049 ) ) ;
#43313=EDGE_LOOP ( 'NONE', ( #50105, #77126, #67865, #35272 ) ) ;
#43314=CARTESIAN_POINT ( 'NONE',  ( 10.64999999999991331, 2.500000000000000000, 6.741600689897071952 ) ) ;
#43315=ORIENTED_EDGE ( 'NONE', *, *, #6656, .T. ) ;
#43316=CARTESIAN_POINT ( 'NONE',  ( 2.499999999999981792, 12.50000000000000000, 4.330127018922196314 ) ) ;
#43317=AXIS2_PLACEMENT_3D ( 'NONE', #51198, #42011, #71455 ) ;
#43318=AXIS2_PLACEMENT_3D ( 'NONE', #90823, #31277, #111081 ) ;
#43319=ORIENTED_EDGE ( 'NONE', *, *, #49612, .F. ) ;
#43320=DIRECTION ( 'NONE',  ( 0.000000000000000000, -0.000000000000000000, 1.000000000000000000 ) ) ;
#43321=CARTESIAN_POINT ( 'NONE',  ( -8.950000000000011724, 2.500000000000000000, -6.148780366869520897 ) ) ;
#43322=ORIENTED_EDGE ( 'NONE', *, *, #6872, .T. ) ;
#43324=ORIENTED_EDGE ( 'NONE', *, *, #107947, .T. ) ;
#43326=DIRECTION ( 'NONE',  ( 0.000000000000000000, -0.9999939076577903929, 0.003490651415223739937 ) ) ;
#43329=CARTESIAN_POINT ( 'NONE',  ( 2.299999999999949640, 12.50000000000000000, -0.3464101615137782364 ) ) ;
#43330=CARTESIAN_POINT ( 'NONE',  ( -2.499999999999996447, 2.500000000000000000, 4.330127018922196314 ) ) ;
#43331=DIRECTION ( 'NONE',  ( 0.000000000000000000, -0.000000000000000000, 1.000000000000000000 ) ) ;
#43332=DIRECTION ( 'NONE',  ( -0.000000000000000000, 1.000000000000000000, -0.000000000000000000 ) ) ;
#43333=CONICAL_SURFACE ( 'NONE', #83045, 0.09999999999999982514, 0.003490658503988666988 ) ;
#43334=EDGE_CURVE ( 'NONE', #13172, #54302, #86944, .T. ) ;
#43335=ORIENTED_EDGE ( 'NONE', *, *, #21180, .F. ) ;
#43336=EDGE_LOOP ( 'NONE', ( #87214, #35800, #74130, #46809 ) ) ;
#43337=DIRECTION ( 'NONE',  ( 0.000000000000000000, 0.000000000000000000, -1.000000000000000000 ) ) ;
#43338=ORIENTED_EDGE ( 'NONE', *, *, #71830, .F. ) ;
#43339=DIRECTION ( 'NONE',  ( 0.000000000000000000, 0.000000000000000000, -1.000000000000000000 ) ) ;
#43340=DIRECTION ( 'NONE',  ( -0.000000000000000000, 1.000000000000000000, -0.000000000000000000 ) ) ;
#43341=CARTESIAN_POINT ( 'NONE',  ( 12.89999999999990266, 2.500000000000000000, -3.537306695894649966 ) ) ;
#43342=VERTEX_POINT ( 'NONE', #95636 ) ;
#43343=VERTEX_POINT ( 'NONE', #124451 ) ;
#43344=ADVANCED_FACE ( 'NONE', ( #5943 ), #103687, .T. ) ;
#43345=FACE_BOUND ( 'NONE', #76191, .T. ) ;
#43346=ORIENTED_EDGE ( 'NONE', *, *, #37422, .F. ) ;
#43348=CARTESIAN_POINT ( 'NONE',  ( -10.40000000000000213, 12.50000000000000000, -0.6928203230275541413 ) ) ;
#43349=DIRECTION ( 'NONE',  ( 0.000000000000000000, 0.000000000000000000, -1.000000000000000000 ) ) ;
#43350=DIRECTION ( 'NONE',  ( 0.000000000000000000, 0.000000000000000000, 1.000000000000000000 ) ) ;
#43351=FACE_OUTER_BOUND ( 'NONE', #8212, .T. ) ;
#43352=AXIS2_PLACEMENT_3D ( 'NONE', #60745, #88917, #49006 ) ;
#43353=FACE_OUTER_BOUND ( 'NONE', #18948, .T. ) ;
#43354=AXIS2_PLACEMENT_3D ( 'NONE', #120695, #93818, #21202 ) ;
#43355=CARTESIAN_POINT ( 'NONE',  ( -3.300000000000028244, 2.500000000000000000, 4.330127018922196314 ) ) ;
#43356=ADVANCED_FACE ( 'NONE', ( #55066 ), #61636, .T. ) ;
#43357=DIRECTION ( 'NONE',  ( -0.000000000000000000, 1.000000000000000000, -0.000000000000000000 ) ) ;
#43358=ADVANCED_FACE ( 'NONE', ( #116554 ), #74153, .T. ) ;
#43359=LINE ( 'NONE', #34835, #48459 ) ;
#43360=FACE_OUTER_BOUND ( 'NONE', #99751, .T. ) ;
#43362=EDGE_CURVE ( 'NONE', #23039, #59349, #30544, .T. ) ;
#43363=CARTESIAN_POINT ( 'NONE',  ( -10.45000000000000107, 12.50000000000000000, 6.495190528383297135 ) ) ;
#43364=AXIS2_PLACEMENT_3D ( 'NONE', #39122, #79655, #79031 ) ;
#43365=VECTOR ( 'NONE', #119081, 1000.000000000000000 ) ;
#43366=EDGE_LOOP ( 'NONE', ( #93382, #65262 ) ) ;
#43367=ORIENTED_EDGE ( 'NONE', *, *, #73653, .T. ) ;
#43368=VECTOR ( 'NONE', #55752, 1000.000000000000000 ) ;
#43369=ORIENTED_EDGE ( 'NONE', *, *, #6045, .F. ) ;
#43370=FACE_OUTER_BOUND ( 'NONE', #4273, .T. ) ;
#43371=EDGE_LOOP ( 'NONE', ( #32431, #124883 ) ) ;
#43372=DIRECTION ( 'NONE',  ( 0.000000000000000000, 0.000000000000000000, -1.000000000000000000 ) ) ;
#43373=ORIENTED_EDGE ( 'NONE', *, *, #18810, .F. ) ;
#43374=ORIENTED_EDGE ( 'NONE', *, *, #67889, .T. ) ;
#43375=ORIENTED_EDGE ( 'NONE', *, *, #52310, .T. ) ;
#43376=CARTESIAN_POINT ( 'NONE',  ( -8.150000000000012790, 2.500000000000000000, -1.818653347947326138 ) ) ;
#43377=AXIS2_PLACEMENT_3D ( 'NONE', #46146, #86054, #93964 ) ;
#43378=AXIS2_PLACEMENT_3D ( 'NONE', #84353, #93531, #54882 ) ;
#43379=VECTOR ( 'NONE', #121240, 1000.000000000000000 ) ;
#43380=LINE ( 'NONE', #101643, #17464 ) ;
#43381=FACE_OUTER_BOUND ( 'NONE', #5634, .T. ) ;
#43382=CARTESIAN_POINT ( 'NONE',  ( -6.249999999999981348, 2.500000000000000000, 2.165063509461097713 ) ) ;
#43383=CARTESIAN_POINT ( 'NONE',  ( 11.04999999999990834, 2.500000000000000000, 1.818653347947321475 ) ) ;
#43384=ORIENTED_EDGE ( 'NONE', *, *, #63860, .F. ) ;
#43385=LINE ( 'NONE', #112114, #83236 ) ;
#43386=ORIENTED_EDGE ( 'NONE', *, *, #95510, .F. ) ;
#43387=ORIENTED_EDGE ( 'NONE', *, *, #24810, .T. ) ;
#43388=EDGE_LOOP ( 'NONE', ( #59807, #18497, #123211, #39543 ) ) ;
#43389=AXIS2_PLACEMENT_3D ( 'NONE', #71184, #87117, #127061 ) ;
#43390=DIRECTION ( 'NONE',  ( 0.000000000000000000, -0.000000000000000000, 1.000000000000000000 ) ) ;
#43391=EDGE_LOOP ( 'NONE', ( #109918, #106920, #53638, #71156 ) ) ;
#43392=ORIENTED_EDGE ( 'NONE', *, *, #124594, .F. ) ;
#43393=EDGE_LOOP ( 'NONE', ( #73718, #15096, #55299, #25119 ) ) ;
#43394=AXIS2_PLACEMENT_3D ( 'NONE', #17571, #77777, #28057 ) ;
#43395=DIRECTION ( 'NONE',  ( 0.000000000000000000, 1.000000000000000000, 0.000000000000000000 ) ) ;
#43396=CARTESIAN_POINT ( 'NONE',  ( -2.499999999999996447, 12.50000000000000000, 4.330127018922196314 ) ) ;
#43397=DIRECTION ( 'NONE',  ( -0.000000000000000000, 1.000000000000000000, -0.000000000000000000 ) ) ;
#43398=CIRCLE ( 'NONE', #62173, 0.06509327318403745899 ) ;
#43399=FACE_OUTER_BOUND ( 'NONE', #125435, .T. ) ;
#43400=CARTESIAN_POINT ( 'NONE',  ( 4.349999999999941025, 2.500000000000000000, -6.148780366869526226 ) ) ;
#43401=EDGE_CURVE ( 'NONE', #113534, #70253, #78367, .T. ) ;
#43402=PLANE ( 'NONE',  #77935 ) ;
#43403=EDGE_CURVE ( 'NONE', #20780, #112974, #13487, .T. ) ;
#43404=AXIS2_PLACEMENT_3D ( 'NONE', #93246, #74892, #101774 ) ;
#43405=ADVANCED_FACE ( 'NONE', ( #126387 ), #76643, .T. ) ;
#43406=PLANE ( 'NONE',  #24107 ) ;
#43407=AXIS2_PLACEMENT_3D ( 'NONE', #40280, #48819, #99850 ) ;
#43408=ORIENTED_EDGE ( 'NONE', *, *, #74525, .T. ) ;
#43409=AXIS2_PLACEMENT_3D ( 'NONE', #100381, #128580, #79462 ) ;
#43410=AXIS2_PLACEMENT_3D ( 'NONE', #108623, #117134, #48419 ) ;
#43411=DIRECTION ( 'NONE',  ( 0.000000000000000000, 0.000000000000000000, 1.000000000000000000 ) ) ;
#43412=ORIENTED_EDGE ( 'NONE', *, *, #89334, .F. ) ;
#43413=FACE_OUTER_BOUND ( 'NONE', #80768, .T. ) ;
#43414=EDGE_CURVE ( 'NONE', #93998, #56130, #76215, .T. ) ;
#43415=ORIENTED_EDGE ( 'NONE', *, *, #34003, .F. ) ;
#43416=CONICAL_SURFACE ( 'NONE', #49676, 0.09999999999999999167, 0.003490658503988666988 ) ;
#43417=ADVANCED_FACE ( 'NONE', ( #45250 ), #38665, .T. ) ;
#43418=VERTEX_POINT ( 'NONE', #49780 ) ;
#43419=PLANE ( 'NONE',  #30234 ) ;
#43420=ADVANCED_FACE ( 'NONE', ( #117175 ), #89683, .T. ) ;
#43421=CARTESIAN_POINT ( 'NONE',  ( 2.499999999999945377, 2.500000000000000000, 5.022947341949748790 ) ) ;
#43422=EDGE_CURVE ( 'NONE', #781, #64023, #111814, .T. ) ;
#43423=CIRCLE ( 'NONE', #76854, 0.09999999999999982514 ) ;
#43424=CIRCLE ( 'NONE', #10047, 0.06509327318403745899 ) ;
#43425=EDGE_CURVE ( 'NONE', #85131, #83089, #34450, .T. ) ;
#43426=DIRECTION ( 'NONE',  ( 0.000000000000000000, -0.000000000000000000, 1.000000000000000000 ) ) ;
#43427=VERTEX_POINT ( 'NONE', #127044 ) ;
#43428=VERTEX_POINT ( 'NONE', #77917 ) ;
#43429=CARTESIAN_POINT ( 'NONE',  ( -2.700000000000030820, 2.500000000000000000, 0.2464101615137735679 ) ) ;
#43430=CARTESIAN_POINT ( 'NONE',  ( 12.29999999999990479, 2.500000000000000000, -3.983716857408426293 ) ) ;
#43431=DIRECTION ( 'NONE',  ( 0.000000000000000000, 0.000000000000000000, 1.000000000000000000 ) ) ;
#43432=DIRECTION ( 'NONE',  ( 0.000000000000000000, 1.000000000000000000, 0.000000000000000000 ) ) ;
#43433=ADVANCED_FACE ( 'NONE', ( #37375 ), #51176, .T. ) ;
#43434=DIRECTION ( 'NONE',  ( 0.000000000000000000, 1.000000000000000000, 0.000000000000000000 ) ) ;
#43435=ORIENTED_EDGE ( 'NONE', *, *, #54088, .T. ) ;
#43436=CARTESIAN_POINT ( 'NONE',  ( -4.600000000000028066, 2.500000000000000000, -4.922947341949753586 ) ) ;
#43437=CIRCLE ( 'NONE', #80977, 0.1000000000000002554 ) ;
#43438=ORIENTED_EDGE ( 'NONE', *, *, #40155, .T. ) ;
#43439=FACE_OUTER_BOUND ( 'NONE', #28170, .T. ) ;
#43440=CARTESIAN_POINT ( 'NONE',  ( 8.749999999999953815, 2.500000000000000000, -2.165063509461101710 ) ) ;
#43442=LINE ( 'NONE', #64346, #5130 ) ;
#43443=CARTESIAN_POINT ( 'NONE',  ( -11.64999999999999680, 12.50000000000000000, -2.230156782645135394 ) ) ;
#43444=CARTESIAN_POINT ( 'NONE',  ( -7.700000000000016165, 2.500000000000000000, -3.983716857408426293 ) ) ;
#43445=DIRECTION ( 'NONE',  ( 0.000000000000000000, 1.000000000000000000, 0.000000000000000000 ) ) ;
#43446=ORIENTED_EDGE ( 'NONE', *, *, #123424, .T. ) ;
#43447=VECTOR ( 'NONE', #93426, 1000.000000000000000 ) ;
#43448=FACE_OUTER_BOUND ( 'NONE', #76335, .T. ) ;
#43449=CIRCLE ( 'NONE', #64352, 0.06509327318403745899 ) ;
#43450=FACE_OUTER_BOUND ( 'NONE', #72644, .T. ) ;
#43451=LINE ( 'NONE', #44073, #89440 ) ;
#43452=ORIENTED_EDGE ( 'NONE', *, *, #93055, .T. ) ;
#43453=DIRECTION ( 'NONE',  ( 0.000000000000000000, 1.000000000000000000, 0.000000000000000000 ) ) ;
#43454=CONICAL_SURFACE ( 'NONE', #66415, 0.1000000000000000056, 0.003490658503988666988 ) ;
#43455=EDGE_CURVE ( 'NONE', #44343, #84404, #7516, .T. ) ;
#43456=CONICAL_SURFACE ( 'NONE', #50007, 0.1000000000000000472, 0.003490658503988666988 ) ;
#43457=EDGE_LOOP ( 'NONE', ( #61365, #96149 ) ) ;
#43458=FACE_OUTER_BOUND ( 'NONE', #36362, .T. ) ;
#43459=EDGE_LOOP ( 'NONE', ( #113729, #111352 ) ) ;
#43460=PLANE ( 'NONE',  #91926 ) ;
#43461=CARTESIAN_POINT ( 'NONE',  ( -3.150000000000030109, 12.50000000000000000, 1.753560074763284016 ) ) ;
#43463=ORIENTED_EDGE ( 'NONE', *, *, #62451, .F. ) ;
#43464=AXIS2_PLACEMENT_3D ( 'NONE', #41255, #121721, #50404 ) ;
#43465=DIRECTION ( 'NONE',  ( -0.000000000000000000, -1.000000000000000000, -0.000000000000000000 ) ) ;
#43466=CARTESIAN_POINT ( 'NONE',  ( 11.64999999999990798, 2.500000000000000000, 5.802370205355744659 ) ) ;
#43467=CIRCLE ( 'NONE', #60193, 0.06509327318403745899 ) ;
#43468=ORIENTED_EDGE ( 'NONE', *, *, #55250, .F. ) ;
#43469=VECTOR ( 'NONE', #43307, 1000.000000000000000 ) ;
#43470=ORIENTED_EDGE ( 'NONE', *, *, #14410, .F. ) ;
#43471=EDGE_LOOP ( 'NONE', ( #56566, #36665 ) ) ;
#43472=DIRECTION ( 'NONE',  ( 0.000000000000000000, 1.000000000000000000, 0.000000000000000000 ) ) ;
#43473=CARTESIAN_POINT ( 'NONE',  ( -5.650000000000019895, 12.50000000000000000, 6.776507416713035248 ) ) ;
#43475=VERTEX_POINT ( 'NONE', #77281 ) ;
#43476=CIRCLE ( 'NONE', #53927, 0.06509327318403745899 ) ;
#43478=FACE_OUTER_BOUND ( 'NONE', #8643, .T. ) ;
#43479=CIRCLE ( 'NONE', #62353, 0.09999999999999982514 ) ;
#43480=ORIENTED_EDGE ( 'NONE', *, *, #2173, .T. ) ;
#43481=DIRECTION ( 'NONE',  ( -0.000000000000000000, 1.000000000000000000, -0.000000000000000000 ) ) ;
#43482=CARTESIAN_POINT ( 'NONE',  ( 0.8499999999999536815, 12.50000000000000000, 6.495190528383297135 ) ) ;
#43483=CONICAL_SURFACE ( 'NONE', #5790, 0.09999999999999982514, 0.003490658503988666988 ) ;
#43484=DIRECTION ( 'NONE',  ( 0.000000000000000000, -0.000000000000000000, 1.000000000000000000 ) ) ;
#43485=CARTESIAN_POINT ( 'NONE',  ( 11.69999999999990870, 12.50000000000000000, 4.265033745738159077 ) ) ;
#43486=DIRECTION ( 'NONE',  ( -0.000000000000000000, -1.000000000000000000, -0.000000000000000000 ) ) ;
#43487=DIRECTION ( 'NONE',  ( 0.000000000000000000, 1.000000000000000000, 0.000000000000000000 ) ) ;
#43488=DIRECTION ( 'NONE',  ( 0.000000000000000000, 1.000000000000000000, 0.000000000000000000 ) ) ;
#43489=AXIS2_PLACEMENT_3D ( 'NONE', #66980, #16591, #85351 ) ;
#43490=AXIS2_PLACEMENT_3D ( 'NONE', #115053, #77087, #25387 ) ;
#43491=EDGE_CURVE ( 'NONE', #67379, #60185, #30137, .T. ) ;
#43492=ORIENTED_EDGE ( 'NONE', *, *, #45182, .F. ) ;
#43493=EDGE_LOOP ( 'NONE', ( #3715, #16985, #79161, #25953 ) ) ;
#43494=ORIENTED_EDGE ( 'NONE', *, *, #117673, .T. ) ;
#43495=EDGE_LOOP ( 'NONE', ( #114603, #84715 ) ) ;
#43496=DIRECTION ( 'NONE',  ( -4.274815082592931898E-19, -0.9999939076577903929, -0.003490651415223739937 ) ) ;
#43497=DIRECTION ( 'NONE',  ( -0.000000000000000000, 1.000000000000000000, -0.000000000000000000 ) ) ;
#43498=CARTESIAN_POINT ( 'NONE',  ( 8.949999999999921130, 2.500000000000000000, -6.741600689897078169 ) ) ;
#43500=VERTEX_POINT ( 'NONE', #70047 ) ;
#43501=EDGE_CURVE ( 'NONE', #76876, #108726, #38000, .T. ) ;
#43502=FACE_BOUND ( 'NONE', #97209, .T. ) ;
#43503=EDGE_CURVE ( 'NONE', #92053, #69317, #67425, .T. ) ;
#43504=DIRECTION ( 'NONE',  ( 0.000000000000000000, 0.000000000000000000, 1.000000000000000000 ) ) ;
#43505=CARTESIAN_POINT ( 'NONE',  ( -8.150000000000012790, 2.500000000000000000, -1.818653347947326138 ) ) ;
#43506=DIRECTION ( 'NONE',  ( 0.000000000000000000, 0.000000000000000000, 1.000000000000000000 ) ) ;
#43507=CIRCLE ( 'NONE', #12166, 0.06509327318403745899 ) ;
#43508=AXIS2_PLACEMENT_3D ( 'NONE', #2691, #124420, #82573 ) ;
#43509=CARTESIAN_POINT ( 'NONE',  ( 7.099999999999928590, 2.500000000000000000, -5.022947341949754119 ) ) ;
#43510=CARTESIAN_POINT ( 'NONE',  ( 21.34481565588170682, -0.7053969147713181620, 2.184679923000722113 ) ) ;
#43511=EDGE_CURVE ( 'NONE', #40817, #25459, #108025, .T. ) ;
#43512=DIRECTION ( 'NONE',  ( 0.000000000000000000, -0.000000000000000000, 1.000000000000000000 ) ) ;
#43513=EDGE_CURVE ( 'NONE', #1730, #65247, #124321, .T. ) ;
#43514=CARTESIAN_POINT ( 'NONE',  ( -5.600000000000023626, 2.500000000000000000, -4.776537180435977525 ) ) ;
#43515=DIRECTION ( 'NONE',  ( -0.000000000000000000, 1.000000000000000000, -0.000000000000000000 ) ) ;
#43517=FACE_OUTER_BOUND ( 'NONE', #39166, .T. ) ;
#43518=EDGE_CURVE ( 'NONE', #43610, #49071, #30257, .T. ) ;
#43520=ORIENTED_EDGE ( 'NONE', *, *, #25914, .F. ) ;
#43521=ORIENTED_EDGE ( 'NONE', *, *, #64077, .T. ) ;
#43522=EDGE_LOOP ( 'NONE', ( #69444, #99, #6491, #107006 ) ) ;
#43523=ORIENTED_EDGE ( 'NONE', *, *, #101590, .F. ) ;
#43524=EDGE_LOOP ( 'NONE', ( #35175, #99250 ) ) ;
#43525=ORIENTED_EDGE ( 'NONE', *, *, #65456, .T. ) ;
#43526=DIRECTION ( 'NONE',  ( 0.000000000000000000, 1.000000000000000000, 0.000000000000000000 ) ) ;
#43527=VERTEX_POINT ( 'NONE', #87091 ) ;
#43528=EDGE_CURVE ( 'NONE', #40454, #97017, #84616, .T. ) ;
#43529=ORIENTED_EDGE ( 'NONE', *, *, #55883, .F. ) ;
#43530=ADVANCED_FACE ( 'NONE', ( #88368 ), #109658, .T. ) ;
#43531=CARTESIAN_POINT ( 'NONE',  ( 14.37945523803864845, -1.500000000000095701, 7.667852710427166762 ) ) ;
#43532=CIRCLE ( 'NONE', #127145, 0.1000000000000002554 ) ;
#43533=DIRECTION ( 'NONE',  ( 0.000000000000000000, 0.000000000000000000, 1.000000000000000000 ) ) ;
#43534=DIRECTION ( 'NONE',  ( 0.000000000000000000, 0.000000000000000000, -1.000000000000000000 ) ) ;
#43535=CIRCLE ( 'NONE', #37270, 0.09999999999999982514 ) ;
#43536=ORIENTED_EDGE ( 'NONE', *, *, #82551, .F. ) ;
#43537=FACE_OUTER_BOUND ( 'NONE', #22414, .T. ) ;
#43538=AXIS2_PLACEMENT_3D ( 'NONE', #72196, #81376, #42756 ) ;
#43539=ORIENTED_EDGE ( 'NONE', *, *, #70349, .F. ) ;
#43540=CIRCLE ( 'NONE', #81175, 0.06509327318403743123 ) ;
#43541=ORIENTED_EDGE ( 'NONE', *, *, #77508, .F. ) ;
#43542=DIRECTION ( 'NONE',  ( -0.000000000000000000, -1.000000000000000000, -0.000000000000000000 ) ) ;
#43543=LINE ( 'NONE', #103086, #60852 ) ;
#43544=VERTEX_POINT ( 'NONE', #99518 ) ;
#43545=CIRCLE ( 'NONE', #118831, 0.09999999999999999167 ) ;
#43546=ORIENTED_EDGE ( 'NONE', *, *, #50168, .F. ) ;
#43547=PLANE ( 'NONE',  #33876 ) ;
#43548=CIRCLE ( 'NONE', #18391, 0.1000000000000002554 ) ;
#43549=DIRECTION ( 'NONE',  ( 0.000000000000000000, -0.000000000000000000, 1.000000000000000000 ) ) ;
#43550=DIRECTION ( 'NONE',  ( 0.000000000000000000, 1.000000000000000000, 0.000000000000000000 ) ) ;
#43551=DIRECTION ( 'NONE',  ( -4.274815082592931898E-19, -0.9999939076577903929, -0.003490651415223739937 ) ) ;
#43552=LINE ( 'NONE', #124680, #2234 ) ;
#43553=ADVANCED_FACE ( 'NONE', ( #128994 ), #63971, .T. ) ;
#43554=ORIENTED_EDGE ( 'NONE', *, *, #36580, .T. ) ;
#43555=EDGE_CURVE ( 'NONE', #19960, #72741, #40720, .T. ) ;
#43556=DIRECTION ( 'NONE',  ( 0.000000000000000000, 1.000000000000000000, 0.000000000000000000 ) ) ;
#43557=CIRCLE ( 'NONE', #110428, 0.1000000000000002554 ) ;
#43558=EDGE_LOOP ( 'NONE', ( #106374, #30092, #103326, #41650 ) ) ;
#43559=PLANE ( 'NONE',  #29484 ) ;
#43560=ADVANCED_FACE ( 'NONE', ( #1294 ), #1932, .T. ) ;
#43561=EDGE_LOOP ( 'NONE', ( #92880, #120324, #110891, #69280 ) ) ;
#43562=CARTESIAN_POINT ( 'NONE',  ( 6.249999999999932498, 12.50000000000000000, 5.802370205355744659 ) ) ;
#43563=CARTESIAN_POINT ( 'NONE',  ( 8.749999999999921840, 12.50000000000000000, -5.802370205355749988 ) ) ;
#43564=CIRCLE ( 'NONE', #104176, 0.06509327318403745899 ) ;
#43566=ADVANCED_FACE ( 'NONE', ( #32069 ), #71987, .T. ) ;
#43567=DIRECTION ( 'NONE',  ( 0.000000000000000000, 1.000000000000000000, 0.000000000000000000 ) ) ;
#43568=ORIENTED_EDGE ( 'NONE', *, *, #75141, .T. ) ;
#43569=EDGE_CURVE ( 'NONE', #84139, #114467, #30783, .T. ) ;
#43570=DIRECTION ( 'NONE',  ( 0.000000000000000000, 0.000000000000000000, -1.000000000000000000 ) ) ;
#43571=AXIS2_PLACEMENT_3D ( 'NONE', #68664, #9096, #47112 ) ;
#43572=EDGE_CURVE ( 'NONE', #41344, #27533, #49124, .T. ) ;
#43574=CARTESIAN_POINT ( 'NONE',  ( 6.049999999999932321, 2.500000000000000000, -1.918653347947326004 ) ) ;
#43575=ORIENTED_EDGE ( 'NONE', *, *, #99348, .T. ) ;
#43576=ORIENTED_EDGE ( 'NONE', *, *, #12546, .F. ) ;
#43577=ORIENTED_EDGE ( 'NONE', *, *, #23427, .F. ) ;
#43578=CARTESIAN_POINT ( 'NONE',  ( 6.249999999999930722, 2.500000000000000000, 7.288010851410849256 ) ) ;
#43579=CARTESIAN_POINT ( 'NONE',  ( 7.099999999999928590, 2.500000000000000000, 3.637306695894644726 ) ) ;
#43581=DIRECTION ( 'NONE',  ( 0.000000000000000000, 0.000000000000000000, 1.000000000000000000 ) ) ;
#43582=CIRCLE ( 'NONE', #18509, 0.09999999999999982514 ) ;
#43583=ADVANCED_FACE ( 'NONE', ( #123014 ), #3241, .T. ) ;
#43585=CIRCLE ( 'NONE', #10206, 0.06509327318403743123 ) ;
#43586=PLANE ( 'NONE',  #90729 ) ;
#43587=DIRECTION ( 'NONE',  ( 0.000000000000000000, 0.000000000000000000, -1.000000000000000000 ) ) ;
#43588=CIRCLE ( 'NONE', #125141, 0.06509327318403745899 ) ;
#43589=ORIENTED_EDGE ( 'NONE', *, *, #17085, .F. ) ;
#43590=CARTESIAN_POINT ( 'NONE',  ( 11.24999999999990941, 12.50000000000000000, -1.472243186433550122 ) ) ;
#43591=ORIENTED_EDGE ( 'NONE', *, *, #33148, .T. ) ;
#43592=CARTESIAN_POINT ( 'NONE',  ( 9.399999999999915090, 12.50000000000000000, 3.983716857408420964 ) ) ;
#43593=VECTOR ( 'NONE', #118329, 1000.000000000000000 ) ;
#43594=PLANE ( 'NONE',  #18014 ) ;
#43596=DIRECTION ( 'NONE',  ( 0.000000000000000000, -0.9999939076577903929, 0.003490651415223739937 ) ) ;
#43597=DIRECTION ( 'NONE',  ( -4.274815082592931898E-19, -0.9999939076577903929, -0.003490651415223739937 ) ) ;
#43598=EDGE_LOOP ( 'NONE', ( #87800, #120110 ) ) ;
#43599=AXIS2_PLACEMENT_3D ( 'NONE', #33665, #74232, #15284 ) ;
#43600=DIRECTION ( 'NONE',  ( -0.000000000000000000, -1.000000000000000000, -0.000000000000000000 ) ) ;
#43601=DIRECTION ( 'NONE',  ( -4.274815082592931898E-19, -0.9999939076577903929, -0.003490651415223739937 ) ) ;
#43602=EDGE_LOOP ( 'NONE', ( #47999, #127862 ) ) ;
#43603=VERTEX_POINT ( 'NONE', #103373 ) ;
#43604=DIRECTION ( 'NONE',  ( -0.000000000000000000, -1.000000000000000000, -0.000000000000000000 ) ) ;
#43605=ADVANCED_FACE ( 'NONE', ( #113176 ), #95171, .T. ) ;
#43606=EDGE_LOOP ( 'NONE', ( #129217, #57922, #17838, #72094 ) ) ;
#43607=ORIENTED_EDGE ( 'NONE', *, *, #64475, .T. ) ;
#43608=DIRECTION ( 'NONE',  ( 0.000000000000000000, -0.000000000000000000, 1.000000000000000000 ) ) ;
#43609=CIRCLE ( 'NONE', #116740, 0.06509327318403745899 ) ;
#43610=VERTEX_POINT ( 'NONE', #60864 ) ;
#43611=CARTESIAN_POINT ( 'NONE',  ( 17.33812564108800203, 2.538896947916920777, -5.379288978441866931 ) ) ;
#43612=FACE_OUTER_BOUND ( 'NONE', #101001, .T. ) ;
#43613=DIRECTION ( 'NONE',  ( 0.000000000000000000, 0.000000000000000000, 1.000000000000000000 ) ) ;
#43614=ORIENTED_EDGE ( 'NONE', *, *, #33975, .F. ) ;
#43615=CIRCLE ( 'NONE', #49881, 0.06509327318403745899 ) ;
#43616=CONICAL_SURFACE ( 'NONE', #24818, 0.1000000000000000472, 0.003490658503988666988 ) ;
#43617=AXIS2_PLACEMENT_3D ( 'NONE', #112441, #51591, #83626 ) ;
#43618=LINE ( 'NONE', #63885, #123562 ) ;
#43619=CARTESIAN_POINT ( 'NONE',  ( -10.85000000000000142, 2.500000000000000000, 2.165063509461097713 ) ) ;
#43621=CARTESIAN_POINT ( 'NONE',  ( 11.24999999999991118, 2.500000000000000000, -2.857883832488653741 ) ) ;
#43622=EDGE_CURVE ( 'NONE', #43976, #100575, #47058, .T. ) ;
#43623=CARTESIAN_POINT ( 'NONE',  ( 17.27571223834416969, -2.230085210383244476, 5.047251339833896289 ) ) ;
#43624=AXIS2_PLACEMENT_3D ( 'NONE', #108379, #90013, #116893 ) ;
#43625=VERTEX_POINT ( 'NONE', #22248 ) ;
#43626=CIRCLE ( 'NONE', #77061, 0.06509327318403745899 ) ;
#43627=ORIENTED_EDGE ( 'NONE', *, *, #12136, .F. ) ;
#43628=AXIS2_PLACEMENT_3D ( 'NONE', #77460, #31593, #80701 ) ;
#43629=EDGE_LOOP ( 'NONE', ( #10252, #44683, #104120, #115717 ) ) ;
#43630=VERTEX_POINT ( 'NONE', #31416 ) ;
#43631=DIRECTION ( 'NONE',  ( 0.000000000000000000, 1.000000000000000000, 0.000000000000000000 ) ) ;
#43632=CARTESIAN_POINT ( 'NONE',  ( -10.20000000000000639, 12.50000000000000000, -3.983716857408421852 ) ) ;
#43633=CARTESIAN_POINT ( 'NONE',  ( -14.34999999999998543, 12.50000000000000000, -1.753560074763286236 ) ) ;
#43634=FACE_BOUND ( 'NONE', #10117, .T. ) ;
#43635=ORIENTED_EDGE ( 'NONE', *, *, #102641, .F. ) ;
#43637=CIRCLE ( 'NONE', #116768, 0.1000000000000002554 ) ;
#43638=FACE_OUTER_BOUND ( 'NONE', #68285, .T. ) ;
#43639=CARTESIAN_POINT ( 'NONE',  ( 9.549999999999915445, 2.500000000000000000, -2.165063509461101710 ) ) ;
#43640=AXIS2_PLACEMENT_3D ( 'NONE', #128262, #108602, #9110 ) ;
#43641=DIRECTION ( 'NONE',  ( -0.000000000000000000, -1.000000000000000000, -0.000000000000000000 ) ) ;
#43642=FACE_OUTER_BOUND ( 'NONE', #111596, .T. ) ;
#43643=DIRECTION ( 'NONE',  ( -0.000000000000000000, -1.000000000000000000, -0.000000000000000000 ) ) ;
#43644=VECTOR ( 'NONE', #6141, 1000.000000000000000 ) ;
#43645=DIRECTION ( 'NONE',  ( -0.000000000000000000, -1.000000000000000000, -0.000000000000000000 ) ) ;
#43646=ADVANCED_FACE ( 'NONE', ( #41887 ), #13027, .T. ) ;
#43647=ORIENTED_EDGE ( 'NONE', *, *, #61499, .T. ) ;
#43648=VERTEX_POINT ( 'NONE', #62172 ) ;
#43649=ORIENTED_EDGE ( 'NONE', *, *, #53415, .F. ) ;
#43650=ORIENTED_EDGE ( 'NONE', *, *, #47946, .F. ) ;
#43651=ORIENTED_EDGE ( 'NONE', *, *, #5932, .T. ) ;
#43652=CIRCLE ( 'NONE', #10192, 0.06509327318403745899 ) ;
#43653=DIRECTION ( 'NONE',  ( 0.000000000000000000, 1.000000000000000000, 0.000000000000000000 ) ) ;
#43654=LINE ( 'NONE', #2397, #63329 ) ;
#43655=ORIENTED_EDGE ( 'NONE', *, *, #127594, .T. ) ;
#43656=FACE_BOUND ( 'NONE', #82401, .T. ) ;
#43657=CARTESIAN_POINT ( 'NONE',  ( -6.050000000000018474, 12.50000000000000000, 2.511473670974873507 ) ) ;
#43658=ADVANCED_FACE ( 'NONE', ( #92247 ), #51065, .T. ) ;
#43659=CONICAL_SURFACE ( 'NONE', #125212, 0.1000000000000002554, 0.003490658503988666988 ) ;
#43660=ORIENTED_EDGE ( 'NONE', *, *, #122144, .F. ) ;
#43661=EDGE_CURVE ( 'NONE', #96104, #38146, #76292, .T. ) ;
#43662=DIRECTION ( 'NONE',  ( 0.000000000000000000, 1.000000000000000000, 0.000000000000000000 ) ) ;
#43663=ADVANCED_FACE ( 'NONE', ( #21584 ), #128560, .T. ) ;
#43664=DIRECTION ( 'NONE',  ( 0.000000000000000000, 0.000000000000000000, 1.000000000000000000 ) ) ;
#43665=ADVANCED_FACE ( 'NONE', ( #42536 ), #52980, .T. ) ;
#43666=CARTESIAN_POINT ( 'NONE',  ( 11.89999999999990798, 12.50000000000000000, -3.983716857408426293 ) ) ;
#43667=ADVANCED_FACE ( 'NONE', ( #96116 ), #65813, .T. ) ;
#43668=ORIENTED_EDGE ( 'NONE', *, *, #45862, .F. ) ;
#43669=CIRCLE ( 'NONE', #125219, 0.06509327318403745899 ) ;
#43670=AXIS2_PLACEMENT_3D ( 'NONE', #83431, #40944, #72325 ) ;
#43671=DIRECTION ( 'NONE',  ( -0.000000000000000000, -1.000000000000000000, -0.000000000000000000 ) ) ;
#43672=AXIS2_PLACEMENT_3D ( 'NONE', #76597, #6523, #36690 ) ;
#43673=EDGE_LOOP ( 'NONE', ( #66841, #73290 ) ) ;
#43674=ADVANCED_FACE ( 'NONE', ( #83733 ), #124416, .T. ) ;
#43675=VERTEX_POINT ( 'NONE', #45104 ) ;
#43676=EDGE_CURVE ( 'NONE', #88341, #59884, #90966, .T. ) ;
#43677=ORIENTED_EDGE ( 'NONE', *, *, #97135, .T. ) ;
#43678=CARTESIAN_POINT ( 'NONE',  ( -8.350000000000008527, 12.50000000000000000, 5.867463478539781896 ) ) ;
#43679=FACE_OUTER_BOUND ( 'NONE', #107442, .T. ) ;
#43680=CARTESIAN_POINT ( 'NONE',  ( -10.65000000000000213, 12.50000000000000000, 6.841600689897072485 ) ) ;
#43681=AXIS2_PLACEMENT_3D ( 'NONE', #44814, #25151, #34356 ) ;
#43682=VERTEX_POINT ( 'NONE', #105943 ) ;
#43683=EDGE_CURVE ( 'NONE', #11681, #112102, #80515, .T. ) ;
#43684=CARTESIAN_POINT ( 'NONE',  ( 15.59999999999988951, 12.50000000000000000, 0.3464101615137735735 ) ) ;
#43685=ADVANCED_FACE ( 'NONE', ( #95478 ), #84700, .T. ) ;
#43686=DIRECTION ( 'NONE',  ( 0.000000000000000000, -0.9999939076577903929, 0.003490651415223739937 ) ) ;
#43687=EDGE_CURVE ( 'NONE', #126108, #51535, #82569, .T. ) ;
#43688=CONICAL_SURFACE ( 'NONE', #26944, 0.1000000000000002554, 0.003490658503988666988 ) ;
#43689=CARTESIAN_POINT ( 'NONE',  ( 9.349999999999919709, 2.500000000000000000, -6.148780366869526226 ) ) ;
#43692=VERTEX_POINT ( 'NONE', #45743 ) ;
#43693=CIRCLE ( 'NONE', #37424, 0.06509327318403745899 ) ;
#43694=LINE ( 'NONE', #82956, #70421 ) ;
#43695=ADVANCED_FACE ( 'NONE', ( #33986 ), #99288, .T. ) ;
#43696=ORIENTED_EDGE ( 'NONE', *, *, #109256, .F. ) ;
#43697=DIRECTION ( 'NONE',  ( -0.000000000000000000, 1.000000000000000000, -0.000000000000000000 ) ) ;
#43698=CONICAL_SURFACE ( 'NONE', #114674, 0.1000000000000002554, 0.003490658503988666988 ) ;
#43699=AXIS2_PLACEMENT_3D ( 'NONE', #35237, #43772, #52288 ) ;
#43700=ORIENTED_EDGE ( 'NONE', *, *, #29444, .T. ) ;
#43701=ORIENTED_EDGE ( 'NONE', *, *, #82711, .T. ) ;
#43702=DIRECTION ( 'NONE',  ( -0.000000000000000000, -1.000000000000000000, -0.000000000000000000 ) ) ;
#43703=DIRECTION ( 'NONE',  ( 0.000000000000000000, 0.000000000000000000, -1.000000000000000000 ) ) ;
#43704=CARTESIAN_POINT ( 'NONE',  ( 3.149999999999942624, 2.500000000000000000, 6.941600689897073018 ) ) ;
#43705=DIRECTION ( 'NONE',  ( 0.000000000000000000, 1.000000000000000000, 0.000000000000000000 ) ) ;
#43706=LINE ( 'NONE', #123513, #22521 ) ;
#43707=EDGE_LOOP ( 'NONE', ( #104152, #16916, #52197, #55957 ) ) ;
#43708=EDGE_LOOP ( 'NONE', ( #55260, #73291 ) ) ;
#43709=DIRECTION ( 'NONE',  ( 0.000000000000000000, 0.000000000000000000, 1.000000000000000000 ) ) ;
#43710=DIRECTION ( 'NONE',  ( 0.000000000000000000, 0.000000000000000000, 1.000000000000000000 ) ) ;
#43712=AXIS2_PLACEMENT_3D ( 'NONE', #112232, #39164, #79075 ) ;
#43713=VERTEX_POINT ( 'NONE', #85006 ) ;
#43714=ORIENTED_EDGE ( 'NONE', *, *, #128660, .T. ) ;
#43715=CARTESIAN_POINT ( 'NONE',  ( 9.999999999999948486, 12.50000000000000000, 4.330127018922196314 ) ) ;
#43716=EDGE_LOOP ( 'NONE', ( #31128, #4559, #98863, #45338 ) ) ;
#43717=CARTESIAN_POINT ( 'NONE',  ( 6.049999999999932321, 12.50000000000000000, 1.883746621131358934 ) ) ;
#43719=VECTOR ( 'NONE', #106655, 1000.000000000000000 ) ;
#43720=DIRECTION ( 'NONE',  ( -0.000000000000000000, -1.000000000000000000, -0.000000000000000000 ) ) ;
#43721=ORIENTED_EDGE ( 'NONE', *, *, #71565, .F. ) ;
#43722=FACE_OUTER_BOUND ( 'NONE', #37064, .T. ) ;
#43723=DIRECTION ( 'NONE',  ( 0.000000000000000000, 0.000000000000000000, 1.000000000000000000 ) ) ;
#43724=CARTESIAN_POINT ( 'NONE',  ( -1.900000000000035438, 12.50000000000000000, 3.983716857408420076 ) ) ;
#43725=FACE_OUTER_BOUND ( 'NONE', #62927, .T. ) ;
#43726=AXIS2_PLACEMENT_3D ( 'NONE', #21185, #20552, #100400 ) ;
#43727=ORIENTED_EDGE ( 'NONE', *, *, #114252, .T. ) ;
#43728=ADVANCED_FACE ( 'NONE', ( #53625 ), #115999, .T. ) ;
#43729=AXIS2_PLACEMENT_3D ( 'NONE', #114991, #65900, #25322 ) ;
#43730=DIRECTION ( 'NONE',  ( 0.000000000000000000, 0.000000000000000000, -1.000000000000000000 ) ) ;
#43731=CARTESIAN_POINT ( 'NONE',  ( 48.84100846698766674, -2.320798421879386453, 5.300800859560139244 ) ) ;
#43732=EDGE_CURVE ( 'NONE', #78632, #16842, #5789, .T. ) ;
#43733=EDGE_LOOP ( 'NONE', ( #15227, #106097, #14743, #102233 ) ) ;
#43734=VERTEX_POINT ( 'NONE', #85656 ) ;
#43737=DIRECTION ( 'NONE',  ( -0.000000000000000000, 1.000000000000000000, -0.000000000000000000 ) ) ;
#43738=CONICAL_SURFACE ( 'NONE', #116852, 0.09999999999999982514, 0.003490658503988666988 ) ;
#43739=FACE_OUTER_BOUND ( 'NONE', #21249, .T. ) ;
#43740=ADVANCED_FACE ( 'NONE', ( #125568 ), #42879, .T. ) ;
#43741=DIRECTION ( 'NONE',  ( 0.000000000000000000, -0.9999939076577903929, 0.003490651415223739937 ) ) ;
#43742=CIRCLE ( 'NONE', #127349, 0.06509327318403745899 ) ;
#43743=FACE_OUTER_BOUND ( 'NONE', #86615, .T. ) ;
#43744=DIRECTION ( 'NONE',  ( 0.000000000000000000, 1.000000000000000000, 0.000000000000000000 ) ) ;
#43745=LINE ( 'NONE', #24725, #28048 ) ;
#43746=CARTESIAN_POINT ( 'NONE',  ( -13.34999999999999076, 2.500000000000000000, 2.165063509461101265 ) ) ;
#43747=CARTESIAN_POINT ( 'NONE',  ( -3.350000000000028511, 12.50000000000000000, 1.472243186433545459 ) ) ;
#43748=FACE_OUTER_BOUND ( 'NONE', #117776, .T. ) ;
#43749=VERTEX_POINT ( 'NONE', #124941 ) ;
#43750=ORIENTED_EDGE ( 'NONE', *, *, #75759, .F. ) ;
#43751=ORIENTED_EDGE ( 'NONE', *, *, #124846, .F. ) ;
#43752=AXIS2_PLACEMENT_3D ( 'NONE', #46093, #57194, #57852 ) ;
#43753=ORIENTED_EDGE ( 'NONE', *, *, #106270, .T. ) ;
#43754=DIRECTION ( 'NONE',  ( 0.000000000000000000, 0.000000000000000000, 1.000000000000000000 ) ) ;
#43755=DIRECTION ( 'NONE',  ( 0.000000000000000000, 1.000000000000000000, 0.000000000000000000 ) ) ;
#43756=ORIENTED_EDGE ( 'NONE', *, *, #44548, .T. ) ;
#43757=DIRECTION ( 'NONE',  ( -0.000000000000000000, 1.000000000000000000, -0.000000000000000000 ) ) ;
#43758=DIRECTION ( 'NONE',  ( 0.000000000000000000, -0.000000000000000000, 1.000000000000000000 ) ) ;
#43759=DIRECTION ( 'NONE',  ( 0.000000000000000000, -0.000000000000000000, 1.000000000000000000 ) ) ;
#43760=ORIENTED_EDGE ( 'NONE', *, *, #67563, .F. ) ;
#43761=DIRECTION ( 'NONE',  ( 0.000000000000000000, 1.000000000000000000, 0.000000000000000000 ) ) ;
#43762=CIRCLE ( 'NONE', #72986, 0.06509327318403745899 ) ;
#43763=DIRECTION ( 'NONE',  ( -4.274815082592931898E-19, -0.9999939076577903929, -0.003490651415223739937 ) ) ;
#43764=ORIENTED_EDGE ( 'NONE', *, *, #43819, .T. ) ;
#43765=CIRCLE ( 'NONE', #10298, 0.1000000000000002554 ) ;
#43766=ORIENTED_EDGE ( 'NONE', *, *, #49447, .T. ) ;
#43767=EDGE_LOOP ( 'NONE', ( #37433, #122055, #88555, #40105 ) ) ;
#43768=ORIENTED_EDGE ( 'NONE', *, *, #45394, .F. ) ;
#43769=DIRECTION ( 'NONE',  ( 0.000000000000000000, 1.000000000000000000, 0.000000000000000000 ) ) ;
#43770=FACE_OUTER_BOUND ( 'NONE', #9400, .T. ) ;
#43771=DIRECTION ( 'NONE',  ( 0.000000000000000000, 0.000000000000000000, 1.000000000000000000 ) ) ;
#43772=DIRECTION ( 'NONE',  ( -0.000000000000000000, -1.000000000000000000, -0.000000000000000000 ) ) ;
#43773=ORIENTED_EDGE ( 'NONE', *, *, #126989, .T. ) ;
#43774=CIRCLE ( 'NONE', #116892, 0.06509327318403745899 ) ;
#43775=VECTOR ( 'NONE', #73707, 1000.000000000000000 ) ;
#43776=DIRECTION ( 'NONE',  ( 0.000000000000000000, -0.9999939076577903929, 0.003490651415223739937 ) ) ;
#43777=EDGE_CURVE ( 'NONE', #61872, #64688, #17791, .T. ) ;
#43778=ORIENTED_EDGE ( 'NONE', *, *, #34960, .F. ) ;
#43779=CARTESIAN_POINT ( 'NONE',  ( -6.249999999999981348, 2.500000000000000000, 6.595190528383296780 ) ) ;
#43780=CARTESIAN_POINT ( 'NONE',  ( 10.28037028461948488, -1.499999999999745981, -9.136909653556401167 ) ) ;
#43781=CONICAL_SURFACE ( 'NONE', #116898, 0.09999999999999982514, 0.003490658503988666988 ) ;
#43782=DIRECTION ( 'NONE',  ( 0.000000000000000000, 0.000000000000000000, 1.000000000000000000 ) ) ;
#43783=CARTESIAN_POINT ( 'NONE',  ( -3.100000000000028511, 2.500000000000000000, 0.4464101615137736623 ) ) ;
#43784=EDGE_CURVE ( 'NONE', #62169, #107629, #43826, .T. ) ;
#43785=ORIENTED_EDGE ( 'NONE', *, *, #106217, .F. ) ;
#43786=AXIS2_PLACEMENT_3D ( 'NONE', #41161, #121614, #60780 ) ;
#43787=CIRCLE ( 'NONE', #39594, 0.1000000000000002554 ) ;
#43788=EDGE_LOOP ( 'NONE', ( #10722, #83527, #61208, #89765 ) ) ;
#43789=EDGE_LOOP ( 'NONE', ( #119315, #40236, #13636, #7027 ) ) ;
#43790=DIRECTION ( 'NONE',  ( -0.000000000000000000, 1.000000000000000000, -0.000000000000000000 ) ) ;
#43791=CARTESIAN_POINT ( 'NONE',  ( -7.900000000000014566, 2.500000000000000000, -3.637306695894650055 ) ) ;
#43792=ADVANCED_FACE ( 'NONE', ( #84369 ), #104641, .T. ) ;
#43793=CARTESIAN_POINT ( 'NONE',  ( -11.25000000000000000, 2.500000000000000000, -7.188010851410850499 ) ) ;
#43794=FACE_BOUND ( 'NONE', #17645, .T. ) ;
#43795=FACE_OUTER_BOUND ( 'NONE', #106062, .T. ) ;
#43796=CARTESIAN_POINT ( 'NONE',  ( 6.849999999999929479, 2.500000000000000000, -2.411473670974877859 ) ) ;
#43797=LINE ( 'NONE', #5127, #72911 ) ;
#43799=DIRECTION ( 'NONE',  ( 0.000000000000000000, 0.000000000000000000, -1.000000000000000000 ) ) ;
#43800=DIRECTION ( 'NONE',  ( 0.000000000000000000, 1.000000000000000000, 0.000000000000000000 ) ) ;
#43801=ORIENTED_EDGE ( 'NONE', *, *, #27110, .T. ) ;
#43802=AXIS2_PLACEMENT_3D ( 'NONE', #20571, #29741, #120057 ) ;
#43803=CONICAL_SURFACE ( 'NONE', #104420, 0.1000000000000002554, 0.003490658503988666988 ) ;
#43804=CARTESIAN_POINT ( 'NONE',  ( -11.05000000000000249, 12.50000000000000000, -1.818653347947322141 ) ) ;
#43805=EDGE_CURVE ( 'NONE', #7901, #18257, #53325, .T. ) ;
#43806=ORIENTED_EDGE ( 'NONE', *, *, #8794, .T. ) ;
#43807=VERTEX_POINT ( 'NONE', #114470 ) ;
#43808=ORIENTED_EDGE ( 'NONE', *, *, #76632, .F. ) ;
#43809=EDGE_LOOP ( 'NONE', ( #47144, #16955, #111153, #38701 ) ) ;
#43810=DIRECTION ( 'NONE',  ( -0.000000000000000000, -1.000000000000000000, -0.000000000000000000 ) ) ;
#43811=FACE_BOUND ( 'NONE', #7454, .T. ) ;
#43812=CARTESIAN_POINT ( 'NONE',  ( 7.299999999999926104, 2.500000000000000000, 4.576537180435972019 ) ) ;
#43813=VECTOR ( 'NONE', #66900, 1000.000000000000000 ) ;
#43814=EDGE_CURVE ( 'NONE', #110184, #101430, #126478, .T. ) ;
#43815=AXIS2_PLACEMENT_3D ( 'NONE', #80558, #38046, #49178 ) ;
#43816=ORIENTED_EDGE ( 'NONE', *, *, #48549, .T. ) ;
#43817=ADVANCED_FACE ( 'NONE', ( #55561 ), #107688, .T. ) ;
#43818=CARTESIAN_POINT ( 'NONE',  ( 76.45351065597657225, 3.568406926244133803, 6.085611129013356546 ) ) ;
#43819=EDGE_CURVE ( 'NONE', #64996, #113749, #51282, .T. ) ;
#43820=DIRECTION ( 'NONE',  ( -0.000000000000000000, 1.000000000000000000, -0.000000000000000000 ) ) ;
#43821=EDGE_CURVE ( 'NONE', #6862, #740, #128173, .T. ) ;
#43822=CIRCLE ( 'NONE', #68929, 0.06509327318403745899 ) ;
#43823=EDGE_CURVE ( 'NONE', #112245, #35444, #69225, .T. ) ;
#43824=ORIENTED_EDGE ( 'NONE', *, *, #51485, .F. ) ;
#43825=DIRECTION ( 'NONE',  ( 0.000000000000000000, 0.000000000000000000, 1.000000000000000000 ) ) ;
#43826=LINE ( 'NONE', #44446, #128644 ) ;
#43827=AXIS2_PLACEMENT_3D ( 'NONE', #73508, #113441, #24420 ) ;
#43828=AXIS2_PLACEMENT_3D ( 'NONE', #54529, #74838, #55834 ) ;
#43829=EDGE_CURVE ( 'NONE', #110014, #35498, #94446, .T. ) ;
#43830=VERTEX_POINT ( 'NONE', #56817 ) ;
#43831=DIRECTION ( 'NONE',  ( 0.000000000000000000, -0.000000000000000000, 1.000000000000000000 ) ) ;
#43832=EDGE_CURVE ( 'NONE', #110433, #27, #113949, .T. ) ;
#43833=CARTESIAN_POINT ( 'NONE',  ( 11.04999999999991012, 2.500000000000000000, 6.741600689897071952 ) ) ;
#43834=ADVANCED_FACE ( 'NONE', ( #118986 ), #9020, .T. ) ;
#43835=ORIENTED_EDGE ( 'NONE', *, *, #125927, .T. ) ;
#43836=DIRECTION ( 'NONE',  ( 0.000000000000000000, -0.9999939076577903929, 0.003490651415223739937 ) ) ;
#43837=ADVANCED_FACE ( 'NONE', ( #119620 ), #3235, .T. ) ;
#43838=DIRECTION ( 'NONE',  ( 0.000000000000000000, 0.000000000000000000, 1.000000000000000000 ) ) ;
#43839=CARTESIAN_POINT ( 'NONE',  ( -9.350000000000006750, 2.500000000000000000, 1.818653347947321475 ) ) ;
#43840=VECTOR ( 'NONE', #119328, 1000.000000000000000 ) ;
#43841=ORIENTED_EDGE ( 'NONE', *, *, #96541, .T. ) ;
#43842=ORIENTED_EDGE ( 'NONE', *, *, #15496, .T. ) ;
#43843=ADVANCED_FACE ( 'NONE', ( #18844 ), #88205, .T. ) ;
#43844=PLANE ( 'NONE',  #49387 ) ;
#43845=EDGE_CURVE ( 'NONE', #2544, #37147, #45098, .T. ) ;
#43846=ORIENTED_EDGE ( 'NONE', *, *, #128990, .T. ) ;
#43847=FACE_OUTER_BOUND ( 'NONE', #123985, .T. ) ;
#43848=CARTESIAN_POINT ( 'NONE',  ( -7.500000000000016875, 2.500000000000000000, 0.5928203230275495006 ) ) ;
#43849=ORIENTED_EDGE ( 'NONE', *, *, #96639, .T. ) ;
#43850=CARTESIAN_POINT ( 'NONE',  ( 11.44999999999991047, 2.500000000000000000, -2.511473670974877948 ) ) ;
#43851=CARTESIAN_POINT ( 'NONE',  ( 3.949999999999940670, 12.50000000000000000, 1.883746621131358934 ) ) ;
#43852=DIRECTION ( 'NONE',  ( 0.000000000000000000, 1.000000000000000000, 0.000000000000000000 ) ) ;
#43853=CARTESIAN_POINT ( 'NONE',  ( -10.40000000000000391, 2.500000000000000000, -3.637306695894645614 ) ) ;
#43854=DIRECTION ( 'NONE',  ( 0.000000000000000000, 0.000000000000000000, 1.000000000000000000 ) ) ;
#43855=ORIENTED_EDGE ( 'NONE', *, *, #50395, .F. ) ;
#43856=EDGE_LOOP ( 'NONE', ( #128189, #100097, #70920, #64253 ) ) ;
#43857=DIRECTION ( 'NONE',  ( 0.000000000000000000, 0.000000000000000000, -1.000000000000000000 ) ) ;
#43859=ORIENTED_EDGE ( 'NONE', *, *, #78944, .F. ) ;
#43860=ORIENTED_EDGE ( 'NONE', *, *, #36877, .T. ) ;
#43862=VECTOR ( 'NONE', #5825, 1000.000000000000000 ) ;
#43863=DIRECTION ( 'NONE',  ( -0.000000000000000000, -1.000000000000000000, -0.000000000000000000 ) ) ;
#43864=CARTESIAN_POINT ( 'NONE',  ( -0.2000000000000412836, 12.50000000000000000, 4.676537180435972552 ) ) ;
#43865=CARTESIAN_POINT ( 'NONE',  ( -10.85000000000000142, 2.500000000000000000, -5.802370205355746435 ) ) ;
#43867=CIRCLE ( 'NONE', #41815, 0.1000000000000002554 ) ;
#43868=CIRCLE ( 'NONE', #33404, 0.06509327318403745899 ) ;
#43869=CYLINDRICAL_SURFACE ( 'NONE', #9725, 2.000000000000000000 ) ;
#43870=LINE ( 'NONE', #15001, #112920 ) ;
#43871=CARTESIAN_POINT ( 'NONE',  ( -7.300000000000018474, 12.50000000000000000, 0.3464101615137735735 ) ) ;
#43872=DIRECTION ( 'NONE',  ( 0.000000000000000000, 0.000000000000000000, 1.000000000000000000 ) ) ;
#43873=DIRECTION ( 'NONE',  ( 0.000000000000000000, -0.9999939076577903929, 0.003490651415223739937 ) ) ;
#43874=CIRCLE ( 'NONE', #56356, 0.09999999999999999167 ) ;
#43875=DIRECTION ( 'NONE',  ( 0.000000000000000000, -0.000000000000000000, 1.000000000000000000 ) ) ;
#43876=VECTOR ( 'NONE', #38424, 1000.000000000000000 ) ;
#43877=EDGE_LOOP ( 'NONE', ( #80168, #24466, #48954, #34494 ) ) ;
#43878=EDGE_CURVE ( 'NONE', #109968, #112742, #55555, .T. ) ;
#43879=EDGE_CURVE ( 'NONE', #16443, #50744, #68591, .T. ) ;
#43880=CARTESIAN_POINT ( 'NONE',  ( -4.999999999999986677, 12.50000000000000000, 4.330127018922196314 ) ) ;
#43881=ORIENTED_EDGE ( 'NONE', *, *, #59422, .F. ) ;
#43882=ORIENTED_EDGE ( 'NONE', *, *, #25081, .F. ) ;
#43883=DIRECTION ( 'NONE',  ( 0.000000000000000000, 1.000000000000000000, 0.000000000000000000 ) ) ;
#43884=LINE ( 'NONE', #54964, #21891 ) ;
#43885=LINE ( 'NONE', #94248, #115472 ) ;
#43887=DIRECTION ( 'NONE',  ( 0.000000000000000000, 0.000000000000000000, 1.000000000000000000 ) ) ;
#43888=DIRECTION ( 'NONE',  ( -0.000000000000000000, -1.000000000000000000, -0.000000000000000000 ) ) ;
#43889=DIRECTION ( 'NONE',  ( 0.000000000000000000, 0.000000000000000000, 1.000000000000000000 ) ) ;
#43890=VERTEX_POINT ( 'NONE', #39167 ) ;
#43891=CARTESIAN_POINT ( 'NONE',  ( -1.650000000000034772, 12.50000000000000000, 5.802370205355744659 ) ) ;
#43892=CARTESIAN_POINT ( 'NONE',  ( 10.59999999999991260, 2.500000000000000000, 0.4464101615137735513 ) ) ;
#43893=VERTEX_POINT ( 'NONE', #47039 ) ;
#43894=CIRCLE ( 'NONE', #68905, 0.06509327318403745899 ) ;
#43895=AXIS2_PLACEMENT_3D ( 'NONE', #78120, #59794, #57839 ) ;
#43896=VERTEX_POINT ( 'NONE', #28033 ) ;
#43897=ORIENTED_EDGE ( 'NONE', *, *, #101908, .F. ) ;
#43898=VERTEX_POINT ( 'NONE', #108518 ) ;
#43899=DIRECTION ( 'NONE',  ( 0.000000000000000000, 0.000000000000000000, 1.000000000000000000 ) ) ;
#43900=DIRECTION ( 'NONE',  ( 0.000000000000000000, 0.000000000000000000, 1.000000000000000000 ) ) ;
#43901=AXIS2_PLACEMENT_3D ( 'NONE', #34199, #82655, #24368 ) ;
#43902=DIRECTION ( 'NONE',  ( 0.000000000000000000, 0.000000000000000000, -1.000000000000000000 ) ) ;
#43903=DIRECTION ( 'NONE',  ( -0.000000000000000000, 1.000000000000000000, -0.000000000000000000 ) ) ;
#43904=CARTESIAN_POINT ( 'NONE',  ( 4.199999999999938005, 2.500000000000000000, 4.330127018922196314 ) ) ;
#43905=EDGE_LOOP ( 'NONE', ( #120599, #10326, #105791, #2504 ) ) ;
#43906=CARTESIAN_POINT ( 'NONE',  ( 12.29999999999990656, 12.50000000000000000, 4.048810130592458201 ) ) ;
#43907=CARTESIAN_POINT ( 'NONE',  ( -5.200000000000025935, 2.500000000000000000, -3.983716857408426293 ) ) ;
#43908=FACE_OUTER_BOUND ( 'NONE', #11185, .T. ) ;
#43909=VECTOR ( 'NONE', #62940, 1000.000000000000000 ) ;
#43910=DIRECTION ( 'NONE',  ( 0.000000000000000000, 0.000000000000000000, 1.000000000000000000 ) ) ;
#43911=AXIS2_PLACEMENT_3D ( 'NONE', #66907, #6677, #46004 ) ;
#43913=ORIENTED_EDGE ( 'NONE', *, *, #96978, .T. ) ;
#43914=AXIS2_PLACEMENT_3D ( 'NONE', #44578, #113309, #54384 ) ;
#43915=EDGE_LOOP ( 'NONE', ( #90796, #126629 ) ) ;
#43916=ORIENTED_EDGE ( 'NONE', *, *, #95965, .T. ) ;
#43917=CARTESIAN_POINT ( 'NONE',  ( -1.650000000000035660, 2.500000000000000000, 7.188010851410848723 ) ) ;
#43918=AXIS2_PLACEMENT_3D ( 'NONE', #127693, #38704, #39347 ) ;
#43919=VECTOR ( 'NONE', #53102, 1000.000000000000000 ) ;
#43920=CARTESIAN_POINT ( 'NONE',  ( -8.350000000000013856, 2.500000000000000000, -2.165063509461101710 ) ) ;
#43921=DIRECTION ( 'NONE',  ( 0.000000000000000000, -0.9999939076577903929, 0.003490651415223739937 ) ) ;
#43922=VECTOR ( 'NONE', #17011, 1000.000000000000000 ) ;
#43923=ADVANCED_FACE ( 'NONE', ( #79080 ), #68061, .T. ) ;
#43924=ORIENTED_EDGE ( 'NONE', *, *, #91665, .F. ) ;
#43925=FACE_OUTER_BOUND ( 'NONE', #31861, .T. ) ;
#43926=DIRECTION ( 'NONE',  ( -0.000000000000000000, -1.000000000000000000, -0.000000000000000000 ) ) ;
#43927=CARTESIAN_POINT ( 'NONE',  ( -7.300000000000014921, 12.50000000000000000, 4.676537180435972552 ) ) ;
#43928=EDGE_CURVE ( 'NONE', #65883, #101366, #79703, .T. ) ;
#43929=CARTESIAN_POINT ( 'NONE',  ( -4.800000000000022915, 2.500000000000000000, 3.883716857408420431 ) ) ;
#43930=LINE ( 'NONE', #104130, #41529 ) ;
#43932=EDGE_LOOP ( 'NONE', ( #107672, #9610, #69110, #103101 ) ) ;
#43933=EDGE_CURVE ( 'NONE', #3855, #12513, #15730, .T. ) ;
#43935=DIRECTION ( 'NONE',  ( 0.000000000000000000, -0.9999939076577903929, 0.003490651415223739937 ) ) ;
#43936=CARTESIAN_POINT ( 'NONE',  ( -3.550000000000028688, 12.50000000000000000, 6.841600689897072485 ) ) ;
#43937=CARTESIAN_POINT ( 'NONE',  ( -5.650000000000019895, 2.500000000000000000, 1.818653347947321475 ) ) ;
#43939=ORIENTED_EDGE ( 'NONE', *, *, #115017, .T. ) ;
#43940=ORIENTED_EDGE ( 'NONE', *, *, #82073, .F. ) ;
#43941=DIRECTION ( 'NONE',  ( -0.000000000000000000, 1.000000000000000000, -0.000000000000000000 ) ) ;
#43942=CIRCLE ( 'NONE', #85773, 0.1000000000000000472 ) ;
#43943=FACE_OUTER_BOUND ( 'NONE', #55128, .T. ) ;
#43944=DIRECTION ( 'NONE',  ( 0.000000000000000000, 0.000000000000000000, -1.000000000000000000 ) ) ;
#43945=CARTESIAN_POINT ( 'NONE',  ( -10.85000000000000142, 12.50000000000000000, -7.253104124594887736 ) ) ;
#43946=ORIENTED_EDGE ( 'NONE', *, *, #45927, .F. ) ;
#43947=CARTESIAN_POINT ( 'NONE',  ( -12.49999999999999467, 2.500000000000000000, -3.637306695894647390 ) ) ;
#43948=AXIS2_PLACEMENT_3D ( 'NONE', #10747, #40248, #80167 ) ;
#43949=DIRECTION ( 'NONE',  ( -0.000000000000000000, -1.000000000000000000, -0.000000000000000000 ) ) ;
#43950=ORIENTED_EDGE ( 'NONE', *, *, #14789, .T. ) ;
#43951=DIRECTION ( 'NONE',  ( 0.000000000000000000, 0.000000000000000000, 1.000000000000000000 ) ) ;
#43952=EDGE_LOOP ( 'NONE', ( #101332, #116123, #56649, #88820 ) ) ;
#43953=DIRECTION ( 'NONE',  ( 0.000000000000000000, 1.000000000000000000, 0.000000000000000000 ) ) ;
#43954=EDGE_CURVE ( 'NONE', #56674, #125960, #128740, .T. ) ;
#43955=ORIENTED_EDGE ( 'NONE', *, *, #70427, .T. ) ;
#43956=DIRECTION ( 'NONE',  ( 0.000000000000000000, 0.000000000000000000, 1.000000000000000000 ) ) ;
#43957=DIRECTION ( 'NONE',  ( 0.000000000000000000, -0.000000000000000000, 1.000000000000000000 ) ) ;
#43958=ORIENTED_EDGE ( 'NONE', *, *, #79617, .F. ) ;
#43959=ORIENTED_EDGE ( 'NONE', *, *, #66517, .T. ) ;
#43960=EDGE_CURVE ( 'NONE', #86305, #48204, #11629, .T. ) ;
#43963=ADVANCED_FACE ( 'NONE', ( #1775 ), #97318, .T. ) ;
#43964=CARTESIAN_POINT ( 'NONE',  ( -4.293440603042597559E-14, 2.500000000000000000, 5.022947341949748790 ) ) ;
#43966=CARTESIAN_POINT ( 'NONE',  ( -0.4000000000000396572, 12.50000000000000000, 3.637306695894644726 ) ) ;
#43967=DIRECTION ( 'NONE',  ( -0.000000000000000000, 1.000000000000000000, -0.000000000000000000 ) ) ;
#43968=EDGE_CURVE ( 'NONE', #122097, #88713, #122858, .T. ) ;
#43969=ADVANCED_FACE ( 'NONE', ( #81630 ), #12872, .T. ) ;
#43970=CARTESIAN_POINT ( 'NONE',  ( -5.600000000000020073, 12.50000000000000000, -0.2813168883297408329 ) ) ;
#43971=CARTESIAN_POINT ( 'NONE',  ( 0.1999999999999567124, 2.500000000000000000, -3.983716857408426293 ) ) ;
#43972=EDGE_CURVE ( 'NONE', #64387, #97052, #12240, .T. ) ;
#43974=CONICAL_SURFACE ( 'NONE', #23037, 0.09999999999999982514, 0.003490658503988666988 ) ;
#43975=AXIS2_PLACEMENT_3D ( 'NONE', #94520, #55886, #74250 ) ;
#43976=VERTEX_POINT ( 'NONE', #82296 ) ;
#43977=ORIENTED_EDGE ( 'NONE', *, *, #23867, .T. ) ;
#43978=DIRECTION ( 'NONE',  ( 0.000000000000000000, 0.000000000000000000, -1.000000000000000000 ) ) ;
#43979=EDGE_CURVE ( 'NONE', #39644, #15846, #51553, .T. ) ;
#43980=EDGE_LOOP ( 'NONE', ( #16245, #17508 ) ) ;
#43981=DIRECTION ( 'NONE',  ( -0.000000000000000000, 1.000000000000000000, -0.000000000000000000 ) ) ;
#43982=DIRECTION ( 'NONE',  ( 0.000000000000000000, -0.000000000000000000, 1.000000000000000000 ) ) ;
#43983=LINE ( 'NONE', #74074, #906 ) ;
#43984=EDGE_LOOP ( 'NONE', ( #126065, #91114, #60230, #91180 ) ) ;
#43985=ORIENTED_EDGE ( 'NONE', *, *, #66804, .F. ) ;
#43986=FACE_BOUND ( 'NONE', #102002, .T. ) ;
#43987=EDGE_LOOP ( 'NONE', ( #10537, #100154 ) ) ;
#43988=DIRECTION ( 'NONE',  ( 0.000000000000000000, 0.000000000000000000, -1.000000000000000000 ) ) ;
#43989=PLANE ( 'NONE',  #112622 ) ;
#43990=CIRCLE ( 'NONE', #69009, 0.06509327318403741736 ) ;
#43991=ADVANCED_FACE ( 'NONE', ( #90147 ), #126568, .T. ) ;
#43992=VERTEX_POINT ( 'NONE', #20149 ) ;
#43993=DIRECTION ( 'NONE',  ( 0.000000000000000000, 0.000000000000000000, 1.000000000000000000 ) ) ;
#43994=LINE ( 'NONE', #123812, #114228 ) ;
#43995=DIRECTION ( 'NONE',  ( -0.000000000000000000, 1.000000000000000000, -0.000000000000000000 ) ) ;
#43996=DIRECTION ( 'NONE',  ( -0.000000000000000000, -1.000000000000000000, -0.000000000000000000 ) ) ;
#43997=CARTESIAN_POINT ( 'NONE',  ( -5.850000000000022737, 2.500000000000000000, -6.495190528383302464 ) ) ;
#43998=FACE_OUTER_BOUND ( 'NONE', #15073, .T. ) ;
#43999=DIRECTION ( 'NONE',  ( 0.000000000000000000, 0.000000000000000000, 1.000000000000000000 ) ) ;
#44000=DIRECTION ( 'NONE',  ( 0.000000000000000000, 0.000000000000000000, 1.000000000000000000 ) ) ;
#44001=DIRECTION ( 'NONE',  ( 0.000000000000000000, 0.000000000000000000, 1.000000000000000000 ) ) ;
#44002=CIRCLE ( 'NONE', #58664, 0.06509327318403745899 ) ;
#44003=ORIENTED_EDGE ( 'NONE', *, *, #26639, .T. ) ;
#44004=ORIENTED_EDGE ( 'NONE', *, *, #90348, .T. ) ;
#44005=VECTOR ( 'NONE', #73870, 1000.000000000000000 ) ;
#44006=ORIENTED_EDGE ( 'NONE', *, *, #43299, .F. ) ;
#44007=FACE_OUTER_BOUND ( 'NONE', #88919, .T. ) ;
#44008=ORIENTED_EDGE ( 'NONE', *, *, #32768, .T. ) ;
#44009=ORIENTED_EDGE ( 'NONE', *, *, #5950, .F. ) ;
#44010=ORIENTED_EDGE ( 'NONE', *, *, #120975, .F. ) ;
#44011=ORIENTED_EDGE ( 'NONE', *, *, #24324, .F. ) ;
#44012=DIRECTION ( 'NONE',  ( 0.000000000000000000, 0.000000000000000000, 1.000000000000000000 ) ) ;
#44013=AXIS2_PLACEMENT_3D ( 'NONE', #94965, #25547, #65484 ) ;
#44014=DIRECTION ( 'NONE',  ( 0.000000000000000000, -0.000000000000000000, 1.000000000000000000 ) ) ;
#44016=DIRECTION ( 'NONE',  ( 0.000000000000000000, -0.000000000000000000, 1.000000000000000000 ) ) ;
#44017=AXIS2_PLACEMENT_3D ( 'NONE', #83083, #25251, #27199 ) ;
#44018=DIRECTION ( 'NONE',  ( 0.000000000000000000, 1.000000000000000000, 0.000000000000000000 ) ) ;
#44019=FACE_OUTER_BOUND ( 'NONE', #114490, .T. ) ;
#44020=ORIENTED_EDGE ( 'NONE', *, *, #92500, .T. ) ;
#44021=CARTESIAN_POINT ( 'NONE',  ( -8.750000000000005329, 12.50000000000000000, 5.802370205355744659 ) ) ;
#44022=ORIENTED_EDGE ( 'NONE', *, *, #42527, .F. ) ;
#44023=EDGE_LOOP ( 'NONE', ( #27014, #113373, #10610, #94292 ) ) ;
#44024=ADVANCED_FACE ( 'NONE', ( #31903 ), #70138, .T. ) ;
#44025=ORIENTED_EDGE ( 'NONE', *, *, #48495, .F. ) ;
#44026=DIRECTION ( 'NONE',  ( -0.000000000000000000, 1.000000000000000000, -0.000000000000000000 ) ) ;
#44027=ORIENTED_EDGE ( 'NONE', *, *, #46477, .T. ) ;
#44028=VERTEX_POINT ( 'NONE', #101930 ) ;
#44029=VERTEX_POINT ( 'NONE', #3090 ) ;
#44030=EDGE_CURVE ( 'NONE', #25747, #63089, #40908, .T. ) ;
#44032=DIRECTION ( 'NONE',  ( 0.000000000000000000, 0.000000000000000000, 1.000000000000000000 ) ) ;
#44033=DIRECTION ( 'NONE',  ( -0.000000000000000000, -1.000000000000000000, -0.000000000000000000 ) ) ;
#44034=CARTESIAN_POINT ( 'NONE',  ( -8.750000000000012434, 2.500000000000000000, -5.802370205355744659 ) ) ;
#44035=CONICAL_SURFACE ( 'NONE', #52332, 0.1000000000000002554, 0.003490658503988666988 ) ;
#44036=DIRECTION ( 'NONE',  ( 0.000000000000000000, -0.000000000000000000, 1.000000000000000000 ) ) ;
#44037=PLANE ( 'NONE',  #45049 ) ;
#44038=ORIENTED_EDGE ( 'NONE', *, *, #36256, .F. ) ;
#44039=DIRECTION ( 'NONE',  ( 0.000000000000000000, -0.000000000000000000, 1.000000000000000000 ) ) ;
#44040=ORIENTED_EDGE ( 'NONE', *, *, #104818, .F. ) ;
#44041=CARTESIAN_POINT ( 'NONE',  ( -9.550000000000006040, 2.500000000000000000, 2.165063509461097713 ) ) ;
#44042=ORIENTED_EDGE ( 'NONE', *, *, #112270, .T. ) ;
#44043=EDGE_LOOP ( 'NONE', ( #20200, #75284, #28800, #91552 ) ) ;
#44044=DIRECTION ( 'NONE',  ( 0.000000000000000000, -0.9999939076577903929, 0.003490651415223739937 ) ) ;
#44045=CARTESIAN_POINT ( 'NONE',  ( 0.8499999999999553468, 2.500000000000000000, -2.757883832488654097 ) ) ;
#44046=DIRECTION ( 'NONE',  ( -0.000000000000000000, 1.000000000000000000, -0.000000000000000000 ) ) ;
#44047=VERTEX_POINT ( 'NONE', #91455 ) ;
#44048=EDGE_LOOP ( 'NONE', ( #1563, #13483, #68018, #117687 ) ) ;
#44049=FACE_OUTER_BOUND ( 'NONE', #44727, .T. ) ;
#44050=CARTESIAN_POINT ( 'NONE',  ( 2.500000000000002220, -1.500000000000000000, -9.999999999999998224 ) ) ;
#44051=DIRECTION ( 'NONE',  ( -0.000000000000000000, -1.000000000000000000, -0.000000000000000000 ) ) ;
#44052=CARTESIAN_POINT ( 'NONE',  ( 8.749999999999921840, 12.50000000000000000, -5.867463478539787225 ) ) ;
#44053=FACE_OUTER_BOUND ( 'NONE', #86400, .T. ) ;
#44054=EDGE_CURVE ( 'NONE', #6303, #97052, #13677, .T. ) ;
#44055=EDGE_LOOP ( 'NONE', ( #24621, #53521, #112740, #48278 ) ) ;
#44056=EDGE_LOOP ( 'NONE', ( #110938, #94469 ) ) ;
#44058=CONICAL_SURFACE ( 'NONE', #79649, 0.1000000000000002554, 0.003490658503988666988 ) ;
#44059=FACE_OUTER_BOUND ( 'NONE', #73458, .T. ) ;
#44060=EDGE_CURVE ( 'NONE', #123049, #109667, #120304, .T. ) ;
#44061=AXIS2_PLACEMENT_3D ( 'NONE', #109199, #111119, #101337 ) ;
#44062=EDGE_CURVE ( 'NONE', #36337, #126006, #30437, .T. ) ;
#44064=CARTESIAN_POINT ( 'NONE',  ( 13.09999999999990195, 2.500000000000000000, -3.883716857408426648 ) ) ;
#44065=DIRECTION ( 'NONE',  ( 0.000000000000000000, 1.000000000000000000, 0.000000000000000000 ) ) ;
#44066=DIRECTION ( 'NONE',  ( -0.000000000000000000, 1.000000000000000000, -0.000000000000000000 ) ) ;
#44067=EDGE_CURVE ( 'NONE', #51768, #13612, #49222, .T. ) ;
#44068=LINE ( 'NONE', #122633, #122848 ) ;
#44069=EDGE_LOOP ( 'NONE', ( #117088, #6917 ) ) ;
#44070=AXIS2_PLACEMENT_3D ( 'NONE', #109767, #111025, #39760 ) ;
#44071=DIRECTION ( 'NONE',  ( -0.000000000000000000, -1.000000000000000000, -0.000000000000000000 ) ) ;
#44072=FACE_OUTER_BOUND ( 'NONE', #123039, .T. ) ;
#44073=CARTESIAN_POINT ( 'NONE',  ( 4.599999999999939249, 2.500000000000000000, -3.537306695894649966 ) ) ;
#44074=EDGE_CURVE ( 'NONE', #4260, #118169, #120285, .T. ) ;
#44075=ORIENTED_EDGE ( 'NONE', *, *, #32174, .F. ) ;
#44076=EDGE_CURVE ( 'NONE', #98404, #85026, #22124, .T. ) ;
#44077=CARTESIAN_POINT ( 'NONE',  ( -13.54999999999999005, 12.50000000000000000, -1.753560074763286458 ) ) ;
#44078=CIRCLE ( 'NONE', #64986, 0.06509327318403743123 ) ;
#44079=EDGE_LOOP ( 'NONE', ( #12797, #84608 ) ) ;
#44081=DIRECTION ( 'NONE',  ( 0.000000000000000000, 0.000000000000000000, -1.000000000000000000 ) ) ;
#44082=VERTEX_POINT ( 'NONE', #100618 ) ;
#44083=CARTESIAN_POINT ( 'NONE',  ( -8.749999999999971578, 2.500000000000000000, 6.495190528383297135 ) ) ;
#44084=DIRECTION ( 'NONE',  ( -0.000000000000000000, -1.000000000000000000, -0.000000000000000000 ) ) ;
#44085=DIRECTION ( 'NONE',  ( 0.000000000000000000, 0.000000000000000000, -1.000000000000000000 ) ) ;
#44086=AXIS2_PLACEMENT_3D ( 'NONE', #65326, #45713, #116364 ) ;
#44087=ORIENTED_EDGE ( 'NONE', *, *, #106889, .T. ) ;
#44088=DIRECTION ( 'NONE',  ( -4.274815082592931898E-19, -0.9999939076577903929, -0.003490651415223739937 ) ) ;
#44089=CARTESIAN_POINT ( 'NONE',  ( 8.549999999999924327, 12.50000000000000000, -6.906693963081115051 ) ) ;
#44090=CIRCLE ( 'NONE', #48298, 0.06509327318403745899 ) ;
#44091=ORIENTED_EDGE ( 'NONE', *, *, #33166, .F. ) ;
#44092=DIRECTION ( 'NONE',  ( -0.000000000000000000, -1.000000000000000000, -0.000000000000000000 ) ) ;
#44093=ORIENTED_EDGE ( 'NONE', *, *, #112351, .T. ) ;
#44094=ORIENTED_EDGE ( 'NONE', *, *, #55033, .T. ) ;
#44095=DIRECTION ( 'NONE',  ( 0.000000000000000000, 1.000000000000000000, 0.000000000000000000 ) ) ;
#44096=DIRECTION ( 'NONE',  ( -0.000000000000000000, -1.000000000000000000, -0.000000000000000000 ) ) ;
#44097=DIRECTION ( 'NONE',  ( 0.000000000000000000, 0.000000000000000000, 1.000000000000000000 ) ) ;
#44098=EDGE_LOOP ( 'NONE', ( #67815, #920 ) ) ;
#44099=CARTESIAN_POINT ( 'NONE',  ( -2.900000000000030109, 12.50000000000000000, 0.7579135962115869374 ) ) ;
#44100=DIRECTION ( 'NONE',  ( -0.000000000000000000, -1.000000000000000000, -0.000000000000000000 ) ) ;
#44101=ORIENTED_EDGE ( 'NONE', *, *, #64327, .F. ) ;
#44102=EDGE_CURVE ( 'NONE', #124893, #45024, #80998, .T. ) ;
#44103=CARTESIAN_POINT ( 'NONE',  ( -11.05000000000000071, 12.50000000000000000, -6.841600689897075149 ) ) ;
#44104=FACE_OUTER_BOUND ( 'NONE', #33516, .T. ) ;
#44105=VECTOR ( 'NONE', #49199, 1000.000000000000000 ) ;
#44106=CARTESIAN_POINT ( 'NONE',  ( 12.49999999999990408, 2.500000000000000000, -3.737306695894649700 ) ) ;
#44107=EDGE_CURVE ( 'NONE', #30037, #56648, #111072, .T. ) ;
#44108=CARTESIAN_POINT ( 'NONE',  ( -12.49999999999999289, 12.50000000000000000, -5.022947341949751454 ) ) ;
#44109=CARTESIAN_POINT ( 'NONE',  ( -2.900000000000029665, 12.50000000000000000, 4.330127018922196314 ) ) ;
#44110=VECTOR ( 'NONE', #17272, 1000.000000000000000 ) ;
#44111=EDGE_CURVE ( 'NONE', #96649, #53518, #122368, .T. ) ;
#44112=AXIS2_PLACEMENT_3D ( 'NONE', #118222, #28562, #118870 ) ;
#44113=CARTESIAN_POINT ( 'NONE',  ( 0.8499999999999545697, 12.50000000000000000, 2.792790559304612064 ) ) ;
#44114=DIRECTION ( 'NONE',  ( 0.000000000000000000, 0.000000000000000000, -1.000000000000000000 ) ) ;
#44115=ADVANCED_FACE ( 'NONE', ( #124136 ), #63867, .T. ) ;
#44116=EDGE_CURVE ( 'NONE', #39602, #103467, #28371, .T. ) ;
#44117=CIRCLE ( 'NONE', #85953, 0.09999999999999982514 ) ;
#44118=VERTEX_POINT ( 'NONE', #73113 ) ;
#44119=ORIENTED_EDGE ( 'NONE', *, *, #69206, .F. ) ;
#44120=ADVANCED_FACE ( 'NONE', ( #103865 ), #51363, .T. ) ;
#44121=ORIENTED_EDGE ( 'NONE', *, *, #3762, .F. ) ;
#44122=ORIENTED_EDGE ( 'NONE', *, *, #98033, .F. ) ;
#44123=CARTESIAN_POINT ( 'NONE',  ( 26.74601813931273853, 2.978655629156508944, 2.722801754518484163 ) ) ;
#44124=DIRECTION ( 'NONE',  ( 0.000000000000000000, 1.000000000000000000, 0.000000000000000000 ) ) ;
#44125=DIRECTION ( 'NONE',  ( -0.000000000000000000, -1.000000000000000000, -0.000000000000000000 ) ) ;
#44126=ORIENTED_EDGE ( 'NONE', *, *, #101129, .F. ) ;
#44127=FACE_BOUND ( 'NONE', #119524, .T. ) ;
#44128=CARTESIAN_POINT ( 'NONE',  ( 4.149999999999938183, 12.50000000000000000, 7.122917578226811486 ) ) ;
#44129=DIRECTION ( 'NONE',  ( 0.000000000000000000, 1.000000000000000000, 0.000000000000000000 ) ) ;
#44130=ADVANCED_FACE ( 'NONE', ( #65198 ), #105135, .T. ) ;
#44131=DIRECTION ( 'NONE',  ( 0.000000000000000000, 0.000000000000000000, 1.000000000000000000 ) ) ;
#44132=EDGE_CURVE ( 'NONE', #129137, #119917, #101524, .T. ) ;
#44133=DIRECTION ( 'NONE',  ( -0.000000000000000000, 1.000000000000000000, -0.000000000000000000 ) ) ;
#44134=DIRECTION ( 'NONE',  ( 0.9974916312695811804, -0.05217691604167136454, 0.04783319955355744973 ) ) ;
#44135=CARTESIAN_POINT ( 'NONE',  ( 1.899999999999949507, 2.500000000000000000, 3.983716857408420964 ) ) ;
#44136=CARTESIAN_POINT ( 'NONE',  ( 11.44999999999990514, 2.500000000000000000, -6.248780366869526759 ) ) ;
#44137=CARTESIAN_POINT ( 'NONE',  ( 12.69999999999989981, 2.500000000000000000, -0.2464101615137783419 ) ) ;
#44138=DIRECTION ( 'NONE',  ( -0.000000000000000000, -1.000000000000000000, -0.000000000000000000 ) ) ;
#44139=CARTESIAN_POINT ( 'NONE',  ( -7.100000000000018296, 2.500000000000000000, 0.09999999999999761857 ) ) ;
#44140=EDGE_LOOP ( 'NONE', ( #40686, #2796 ) ) ;
#44141=CIRCLE ( 'NONE', #12728, 0.06509327318403745899 ) ;
#44142=VERTEX_POINT ( 'NONE', #23343 ) ;
#44143=ORIENTED_EDGE ( 'NONE', *, *, #22671, .T. ) ;
#44145=ORIENTED_EDGE ( 'NONE', *, *, #102534, .T. ) ;
#44146=ORIENTED_EDGE ( 'NONE', *, *, #19203, .T. ) ;
#44147=CARTESIAN_POINT ( 'NONE',  ( 2.500000000000002220, 1.500000000000000444, -9.999999999999998224 ) ) ;
#44148=EDGE_LOOP ( 'NONE', ( #95281, #71893, #75324, #74533 ) ) ;
#44149=ORIENTED_EDGE ( 'NONE', *, *, #126202, .T. ) ;
#44150=CIRCLE ( 'NONE', #119357, 0.1000000000000002554 ) ;
#44151=AXIS2_PLACEMENT_3D ( 'NONE', #40989, #40334, #21311 ) ;
#44152=DIRECTION ( 'NONE',  ( 0.000000000000000000, 1.000000000000000000, 0.000000000000000000 ) ) ;
#44153=CARTESIAN_POINT ( 'NONE',  ( 9.349999999999916156, 2.500000000000000000, 6.248780366869520542 ) ) ;
#44154=DIRECTION ( 'NONE',  ( 0.000000000000000000, 1.000000000000000000, 0.000000000000000000 ) ) ;
#44155=DIRECTION ( 'NONE',  ( 0.000000000000000000, 1.000000000000000000, 0.000000000000000000 ) ) ;
#44156=ORIENTED_EDGE ( 'NONE', *, *, #106463, .T. ) ;
#44157=LINE ( 'NONE', #127709, #10913 ) ;
#44158=AXIS2_PLACEMENT_3D ( 'NONE', #124737, #80089, #112133 ) ;
#44159=CIRCLE ( 'NONE', #56659, 0.1000000000000002554 ) ;
#44160=EDGE_LOOP ( 'NONE', ( #6944, #79268 ) ) ;
#44161=ORIENTED_EDGE ( 'NONE', *, *, #48272, .T. ) ;
#44162=CARTESIAN_POINT ( 'NONE',  ( -11.24999999999996270, 12.50000000000000000, 6.495190528383297135 ) ) ;
#44163=ORIENTED_EDGE ( 'NONE', *, *, #114205, .T. ) ;
#44164=PLANE ( 'NONE',  #52539 ) ;
#44165=ORIENTED_EDGE ( 'NONE', *, *, #68161, .T. ) ;
#44166=CIRCLE ( 'NONE', #39978, 0.06509327318403745899 ) ;
#44168=EDGE_CURVE ( 'NONE', #119345, #23310, #116093, .T. ) ;
#44170=CARTESIAN_POINT ( 'NONE',  ( -4.350000000000023626, 2.500000000000000000, -1.818653347947325916 ) ) ;
#44171=CARTESIAN_POINT ( 'NONE',  ( 8.549999999999924327, 2.500000000000000000, 1.918653347947321564 ) ) ;
#44173=ORIENTED_EDGE ( 'NONE', *, *, #80200, .F. ) ;
#44174=DIRECTION ( 'NONE',  ( 0.000000000000000000, 1.000000000000000000, 0.000000000000000000 ) ) ;
#44176=DIRECTION ( 'NONE',  ( 0.000000000000000000, -0.000000000000000000, 1.000000000000000000 ) ) ;
#44177=EDGE_LOOP ( 'NONE', ( #88073, #11647 ) ) ;
#44178=CARTESIAN_POINT ( 'NONE',  ( 0.8499999999999536815, 2.500000000000000000, 6.495190528383297135 ) ) ;
#44179=CIRCLE ( 'NONE', #25382, 0.09999999999999982514 ) ;
#44180=AXIS2_PLACEMENT_3D ( 'NONE', #122272, #100046, #109869 ) ;
#44181=CARTESIAN_POINT ( 'NONE',  ( 13.14999999999989733, 2.500000000000000000, -2.411473670974877859 ) ) ;
#44182=PLANE ( 'NONE',  #27910 ) ;
#44183=DIRECTION ( 'NONE',  ( 0.000000000000000000, 0.000000000000000000, 1.000000000000000000 ) ) ;
#44184=ORIENTED_EDGE ( 'NONE', *, *, #116187, .F. ) ;
#44185=CARTESIAN_POINT ( 'NONE',  ( -1.850000000000033396, 12.50000000000000000, -6.841600689897077814 ) ) ;
#44186=DIRECTION ( 'NONE',  ( -0.000000000000000000, 1.000000000000000000, -0.000000000000000000 ) ) ;
#44187=EDGE_LOOP ( 'NONE', ( #4586, #67011 ) ) ;
#44188=EDGE_LOOP ( 'NONE', ( #114230, #103848 ) ) ;
#44189=EDGE_LOOP ( 'NONE', ( #26878, #30303, #96992, #79638 ) ) ;
#44190=DIRECTION ( 'NONE',  ( 0.000000000000000000, 0.000000000000000000, -1.000000000000000000 ) ) ;
#44191=CARTESIAN_POINT ( 'NONE',  ( -12.49999999999999289, 2.500000000000000000, 5.022947341949748790 ) ) ;
#44193=DIRECTION ( 'NONE',  ( -0.000000000000000000, -1.000000000000000000, -0.000000000000000000 ) ) ;
#44194=DIRECTION ( 'NONE',  ( 0.000000000000000000, 0.000000000000000000, 1.000000000000000000 ) ) ;
#44195=FACE_OUTER_BOUND ( 'NONE', #98904, .T. ) ;
#44196=AXIS2_PLACEMENT_3D ( 'NONE', #115006, #34559, #96029 ) ;
#44197=CONICAL_SURFACE ( 'NONE', #102684, 0.09999999999999999167, 0.003490658503988666988 ) ;
#44199=ORIENTED_EDGE ( 'NONE', *, *, #40725, .T. ) ;
#44200=DIRECTION ( 'NONE',  ( 0.000000000000000000, 0.000000000000000000, -1.000000000000000000 ) ) ;
#44201=EDGE_CURVE ( 'NONE', #3627, #61342, #104496, .T. ) ;
#44202=AXIS2_PLACEMENT_3D ( 'NONE', #12358, #52296, #122337 ) ;
#44203=AXIS2_PLACEMENT_3D ( 'NONE', #25970, #65881, #36450 ) ;
#44204=VERTEX_POINT ( 'NONE', #84858 ) ;
#44205=CIRCLE ( 'NONE', #37953, 0.1000000000000002554 ) ;
#44207=LINE ( 'NONE', #65124, #34964 ) ;
#44208=CARTESIAN_POINT ( 'NONE',  ( -3.950000000000026379, 2.500000000000000000, -1.718653347947326049 ) ) ;
#44209=CARTESIAN_POINT ( 'NONE',  ( 4.549999999999935874, 12.50000000000000000, 6.430097255199259010 ) ) ;
#44210=EDGE_CURVE ( 'NONE', #40177, #104598, #35764, .T. ) ;
#44211=ORIENTED_EDGE ( 'NONE', *, *, #75384, .F. ) ;
#44212=CARTESIAN_POINT ( 'NONE',  ( -11.44999999999999751, 2.500000000000000000, 1.818653347947321475 ) ) ;
#44213=DIRECTION ( 'NONE',  ( -0.000000000000000000, -1.000000000000000000, -0.000000000000000000 ) ) ;
#44214=ADVANCED_FACE ( 'NONE', ( #53481 ), #126659, .T. ) ;
#44215=ADVANCED_FACE ( 'NONE', ( #115593 ), #99477, .T. ) ;
#44216=ADVANCED_FACE ( 'NONE', ( #3716 ), #26319, .T. ) ;
#44218=EDGE_CURVE ( 'NONE', #100973, #50751, #118332, .T. ) ;
#44220=FACE_OUTER_BOUND ( 'NONE', #91757, .T. ) ;
#44221=EDGE_LOOP ( 'NONE', ( #58253, #77717, #68080, #107018 ) ) ;
#44222=ORIENTED_EDGE ( 'NONE', *, *, #50176, .T. ) ;
#44223=DIRECTION ( 'NONE',  ( 1.000000000000000000, 0.000000000000000000, 0.000000000000000000 ) ) ;
#44224=ADVANCED_FACE ( 'NONE', ( #113684 ), #51727, .T. ) ;
#44225=EDGE_LOOP ( 'NONE', ( #38272, #85977, #93026, #77857 ) ) ;
#44226=CARTESIAN_POINT ( 'NONE',  ( 16.53754090007008770, 0.4856821978169255649, -6.114873053042312989 ) ) ;
#44227=PLANE ( 'NONE',  #77692 ) ;
#44228=DIRECTION ( 'NONE',  ( 0.000000000000000000, 0.000000000000000000, -1.000000000000000000 ) ) ;
#44229=AXIS2_PLACEMENT_3D ( 'NONE', #104578, #94118, #123560 ) ;
#44230=EDGE_LOOP ( 'NONE', ( #7450, #83441 ) ) ;
#44231=AXIS2_PLACEMENT_3D ( 'NONE', #79458, #20533, #60475 ) ;
#44232=CARTESIAN_POINT ( 'NONE',  ( -9.150000000000005684, 2.500000000000000000, 6.495190528383297135 ) ) ;
#44233=CARTESIAN_POINT ( 'NONE',  ( -6.650000000000018119, 2.500000000000000000, -2.165063509461101710 ) ) ;
#44234=ORIENTED_EDGE ( 'NONE', *, *, #19158, .T. ) ;
#44235=CARTESIAN_POINT ( 'NONE',  ( 7.699999999999923794, 2.500000000000000000, 4.576537180435972019 ) ) ;
#44236=CARTESIAN_POINT ( 'NONE',  ( 11.24999999999990585, 2.500000000000000000, 2.857883832488649301 ) ) ;
#44237=VECTOR ( 'NONE', #107982, 1000.000000000000000 ) ;
#44238=EDGE_LOOP ( 'NONE', ( #37945, #119102, #8784, #48723 ) ) ;
#44239=CIRCLE ( 'NONE', #27501, 0.06509327318403745899 ) ;
#44240=CIRCLE ( 'NONE', #113196, 0.06509327318403745899 ) ;
#44241=ORIENTED_EDGE ( 'NONE', *, *, #96076, .F. ) ;
#44242=ORIENTED_EDGE ( 'NONE', *, *, #15225, .T. ) ;
#44243=CARTESIAN_POINT ( 'NONE',  ( -5.650000000000023448, 12.50000000000000000, -2.511473670974877948 ) ) ;
#44244=CARTESIAN_POINT ( 'NONE',  ( -3.550000000000027356, 2.500000000000000000, 1.718653347947321386 ) ) ;
#44245=CARTESIAN_POINT ( 'NONE',  ( -13.09999999999999254, 2.500000000000000000, -4.776537180435974861 ) ) ;
#44246=FACE_BOUND ( 'NONE', #13918, .T. ) ;
#44249=CARTESIAN_POINT ( 'NONE',  ( -1.900000000000034550, 12.50000000000000000, 4.676537180435972552 ) ) ;
#44250=CARTESIAN_POINT ( 'NONE',  ( 0.7999999999999612976, 2.500000000000000000, 0.09999999999999989453 ) ) ;
#44251=FACE_BOUND ( 'NONE', #102656, .T. ) ;
#44252=AXIS2_PLACEMENT_3D ( 'NONE', #108803, #47982, #57140 ) ;
#44253=DIRECTION ( 'NONE',  ( -0.000000000000000000, -1.000000000000000000, -0.000000000000000000 ) ) ;
#44255=ADVANCED_FACE ( 'NONE', ( #66498 ), #6913, .T. ) ;
#44256=CARTESIAN_POINT ( 'NONE',  ( -2.050000000000032685, 2.500000000000000000, -6.395190528383301931 ) ) ;
#44257=AXIS2_PLACEMENT_3D ( 'NONE', #32384, #61167, #101088 ) ;
#44258=EDGE_CURVE ( 'NONE', #32793, #101221, #60425, .T. ) ;
#44259=CARTESIAN_POINT ( 'NONE',  ( 1.849999999999950573, 2.500000000000000000, -1.818653347947326138 ) ) ;
#44260=EDGE_CURVE ( 'NONE', #69086, #20962, #105727, .T. ) ;
#44261=ORIENTED_EDGE ( 'NONE', *, *, #13337, .F. ) ;
#44262=AXIS2_PLACEMENT_3D ( 'NONE', #97564, #18359, #58308 ) ;
#44263=AXIS2_PLACEMENT_3D ( 'NONE', #31166, #120175, #71071 ) ;
#44264=VERTEX_POINT ( 'NONE', #56665 ) ;
#44265=ORIENTED_EDGE ( 'NONE', *, *, #83602, .F. ) ;
#44266=VERTEX_POINT ( 'NONE', #57993 ) ;
#44267=ORIENTED_EDGE ( 'NONE', *, *, #92410, .T. ) ;
#44268=CARTESIAN_POINT ( 'NONE',  ( -13.74999999999995381, 2.500000000000000000, 2.065063509461101621 ) ) ;
#44269=DIRECTION ( 'NONE',  ( -0.000000000000000000, -1.000000000000000000, -0.000000000000000000 ) ) ;
#44270=ORIENTED_EDGE ( 'NONE', *, *, #42162, .T. ) ;
#44271=EDGE_CURVE ( 'NONE', #126312, #71812, #74429, .T. ) ;
#44272=FACE_BOUND ( 'NONE', #12920, .T. ) ;
#44273=PLANE ( 'NONE',  #77118 ) ;
#44274=EDGE_CURVE ( 'NONE', #71913, #110789, #107866, .T. ) ;
#44275=ADVANCED_FACE ( 'NONE', ( #27874 ), #109939, .T. ) ;
#44276=EDGE_CURVE ( 'NONE', #38503, #48843, #122463, .T. ) ;
#44277=DIRECTION ( 'NONE',  ( 0.000000000000000000, 0.000000000000000000, -1.000000000000000000 ) ) ;
#44278=ORIENTED_EDGE ( 'NONE', *, *, #46574, .T. ) ;
#44279=PLANE ( 'NONE',  #32841 ) ;
#44280=DIRECTION ( 'NONE',  ( 0.000000000000000000, -0.9999939076577903929, 0.003490651415223739937 ) ) ;
#44281=DIRECTION ( 'NONE',  ( 0.000000000000000000, 0.000000000000000000, 1.000000000000000000 ) ) ;
#44282=ORIENTED_EDGE ( 'NONE', *, *, #72073, .F. ) ;
#44283=CARTESIAN_POINT ( 'NONE',  ( 16.56576425164991306, -1.499999999999999334, 6.084390597445976212 ) ) ;
#44284=EDGE_CURVE ( 'NONE', #7925, #43068, #38355, .T. ) ;
#44285=ORIENTED_EDGE ( 'NONE', *, *, #6395, .T. ) ;
#44287=CIRCLE ( 'NONE', #92316, 0.06509327318403745899 ) ;
#44288=ORIENTED_EDGE ( 'NONE', *, *, #28279, .T. ) ;
#44289=AXIS2_PLACEMENT_3D ( 'NONE', #105862, #15530, #45664 ) ;
#44290=DIRECTION ( 'NONE',  ( 0.000000000000000000, 1.000000000000000000, 0.000000000000000000 ) ) ;
#44291=AXIS2_PLACEMENT_3D ( 'NONE', #53215, #44676, #85860 ) ;
#44292=DIRECTION ( 'NONE',  ( 0.000000000000000000, -0.9999939076577903929, 0.003490651415223739937 ) ) ;
#44293=DIRECTION ( 'NONE',  ( 0.000000000000000000, 0.000000000000000000, -1.000000000000000000 ) ) ;
#44294=ORIENTED_EDGE ( 'NONE', *, *, #31119, .F. ) ;
#44295=DIRECTION ( 'NONE',  ( 0.000000000000000000, 0.000000000000000000, -1.000000000000000000 ) ) ;
#44296=FACE_OUTER_BOUND ( 'NONE', #25852, .T. ) ;
#44297=CIRCLE ( 'NONE', #19244, 0.09999999999999982514 ) ;
#44298=AXIS2_PLACEMENT_3D ( 'NONE', #83459, #87773, #84075 ) ;
#44299=FACE_OUTER_BOUND ( 'NONE', #98037, .T. ) ;
#44301=ORIENTED_EDGE ( 'NONE', *, *, #71009, .T. ) ;
#44302=CIRCLE ( 'NONE', #67252, 0.1000000000000000472 ) ;
#44303=CONICAL_SURFACE ( 'NONE', #31800, 0.09999999999999999167, 0.003490658503988666988 ) ;
#44304=CARTESIAN_POINT ( 'NONE',  ( -9.800000000000006040, 12.50000000000000000, -4.611443907251936203 ) ) ;
#44305=ADVANCED_FACE ( 'NONE', ( #110142 ), #47252, .T. ) ;
#44306=EDGE_LOOP ( 'NONE', ( #23478, #104427 ) ) ;
#44307=FACE_OUTER_BOUND ( 'NONE', #50825, .T. ) ;
#44308=CIRCLE ( 'NONE', #35907, 0.06509327318403745899 ) ;
#44309=EDGE_LOOP ( 'NONE', ( #71595, #31269, #125964, #14747 ) ) ;
#44310=EDGE_LOOP ( 'NONE', ( #74762, #38418, #98445, #57228 ) ) ;
#44311=CARTESIAN_POINT ( 'NONE',  ( 0.6499999999999561684, 12.50000000000000000, -2.511473670974877948 ) ) ;
#44312=DIRECTION ( 'NONE',  ( 0.000000000000000000, 0.000000000000000000, 1.000000000000000000 ) ) ;
#44313=DIRECTION ( 'NONE',  ( -0.000000000000000000, -1.000000000000000000, -0.000000000000000000 ) ) ;
#44314=CARTESIAN_POINT ( 'NONE',  ( -2.700000000000030820, 2.500000000000000000, 0.3464101615137735735 ) ) ;
#44315=FACE_OUTER_BOUND ( 'NONE', #47133, .T. ) ;
#44316=ORIENTED_EDGE ( 'NONE', *, *, #128001, .F. ) ;
#44317=VERTEX_POINT ( 'NONE', #77604 ) ;
#44318=CARTESIAN_POINT ( 'NONE',  ( -12.49999999999999289, 2.500000000000000000, -0.7928203230275501223 ) ) ;
#44319=EDGE_CURVE ( 'NONE', #17717, #107010, #80695, .T. ) ;
#44321=DIRECTION ( 'NONE',  ( -0.000000000000000000, -1.000000000000000000, -0.000000000000000000 ) ) ;
#44323=EDGE_LOOP ( 'NONE', ( #13240, #19226 ) ) ;
#44324=CARTESIAN_POINT ( 'NONE',  ( 1.649999999999948841, 12.50000000000000000, 6.430097255199259010 ) ) ;
#44325=AXIS2_PLACEMENT_3D ( 'NONE', #22021, #10249, #1704 ) ;
#44326=ORIENTED_EDGE ( 'NONE', *, *, #81890, .F. ) ;
#44327=DIRECTION ( 'NONE',  ( 0.000000000000000000, -0.000000000000000000, 1.000000000000000000 ) ) ;
#44328=AXIS2_PLACEMENT_3D ( 'NONE', #46604, #16481, #49846 ) ;
#44329=CARTESIAN_POINT ( 'NONE',  ( 9.199999999999915801, 12.50000000000000000, 4.265033745738159077 ) ) ;
#44330=ORIENTED_EDGE ( 'NONE', *, *, #83085, .F. ) ;
#44331=DIRECTION ( 'NONE',  ( 0.000000000000000000, 0.000000000000000000, 1.000000000000000000 ) ) ;
#44333=DIRECTION ( 'NONE',  ( 0.000000000000000000, 0.000000000000000000, 1.000000000000000000 ) ) ;
#44334=EDGE_CURVE ( 'NONE', #88750, #95225, #93210, .T. ) ;
#44335=DIRECTION ( 'NONE',  ( 0.000000000000000000, 0.000000000000000000, 1.000000000000000000 ) ) ;
#44336=CONICAL_SURFACE ( 'NONE', #54794, 0.1000000000000002554, 0.003490658503988666988 ) ;
#44337=ORIENTED_EDGE ( 'NONE', *, *, #4604, .F. ) ;
#44338=AXIS2_PLACEMENT_3D ( 'NONE', #114830, #64449, #14686 ) ;
#44339=VECTOR ( 'NONE', #45343, 1000.000000000000000 ) ;
#44340=DIRECTION ( 'NONE',  ( -0.000000000000000000, -1.000000000000000000, -0.000000000000000000 ) ) ;
#44341=CIRCLE ( 'NONE', #65258, 0.1000000000000002554 ) ;
#44342=DIRECTION ( 'NONE',  ( -0.000000000000000000, -1.000000000000000000, -0.000000000000000000 ) ) ;
#44343=VERTEX_POINT ( 'NONE', #120607 ) ;
#44344=ORIENTED_EDGE ( 'NONE', *, *, #23778, .F. ) ;
#44346=FACE_OUTER_BOUND ( 'NONE', #68780, .T. ) ;
#44347=CARTESIAN_POINT ( 'NONE',  ( 13.94999999999989448, 12.50000000000000000, -2.511473670974877948 ) ) ;
#44348=CARTESIAN_POINT ( 'NONE',  ( -6.050000000000020250, 12.50000000000000000, -2.511473670974877948 ) ) ;
#44349=DIRECTION ( 'NONE',  ( 0.000000000000000000, 0.000000000000000000, 1.000000000000000000 ) ) ;
#44350=AXIS2_PLACEMENT_3D ( 'NONE', #94988, #93059, #34137 ) ;
#44351=CARTESIAN_POINT ( 'NONE',  ( -0.2000000000000339284, 2.500000000000000000, -0.3464101615137759604 ) ) ;
#44352=DIRECTION ( 'NONE',  ( -0.000000000000000000, 1.000000000000000000, -0.000000000000000000 ) ) ;
#44353=CIRCLE ( 'NONE', #56853, 0.06509327318403745899 ) ;
#44354=CARTESIAN_POINT ( 'NONE',  ( -6.850000000000017408, 2.500000000000000000, -1.718653347947325827 ) ) ;
#44355=CIRCLE ( 'NONE', #117481, 0.06509327318403745899 ) ;
#44356=DIRECTION ( 'NONE',  ( 0.000000000000000000, 1.000000000000000000, 0.000000000000000000 ) ) ;
#44357=CIRCLE ( 'NONE', #23424, 0.06509327318403745899 ) ;
#44359=CARTESIAN_POINT ( 'NONE',  ( 5.199999999999935341, 2.500000000000000000, -0.4464101615137783252 ) ) ;
#44360=ORIENTED_EDGE ( 'NONE', *, *, #124628, .T. ) ;
#44361=ORIENTED_EDGE ( 'NONE', *, *, #27347, .T. ) ;
#44362=EDGE_CURVE ( 'NONE', #58785, #103318, #28465, .T. ) ;
#44363=AXIS2_PLACEMENT_3D ( 'NONE', #52334, #90975, #80525 ) ;
#44364=ORIENTED_EDGE ( 'NONE', *, *, #117457, .T. ) ;
#44365=ORIENTED_EDGE ( 'NONE', *, *, #40950, .F. ) ;
#44366=CARTESIAN_POINT ( 'NONE',  ( 6.449999999999930012, 2.500000000000000000, 1.818653347947321475 ) ) ;
#44367=CARTESIAN_POINT ( 'NONE',  ( -2.700000000000030376, 2.500000000000000000, 3.983716857408420964 ) ) ;
#44368=DIRECTION ( 'NONE',  ( 0.000000000000000000, -0.9999939076577903929, 0.003490651415223739937 ) ) ;
#44369=EDGE_CURVE ( 'NONE', #38578, #118512, #51246, .T. ) ;
#44370=ORIENTED_EDGE ( 'NONE', *, *, #54823, .F. ) ;
#44371=CARTESIAN_POINT ( 'NONE',  ( 1.699999999999951994, 2.500000000000000000, -4.330127018922201643 ) ) ;
#44372=DIRECTION ( 'NONE',  ( -0.000000000000000000, 1.000000000000000000, -0.000000000000000000 ) ) ;
#44373=CARTESIAN_POINT ( 'NONE',  ( -10.40000000000000213, 2.500000000000000000, 3.737306695894644371 ) ) ;
#44374=ORIENTED_EDGE ( 'NONE', *, *, #88745, .T. ) ;
#44375=EDGE_CURVE ( 'NONE', #129537, #105720, #97401, .T. ) ;
#44376=EDGE_CURVE ( 'NONE', #66886, #48260, #20059, .T. ) ;
#44377=EDGE_CURVE ( 'NONE', #118758, #110045, #117506, .T. ) ;
#44378=DIRECTION ( 'NONE',  ( 0.000000000000000000, 0.000000000000000000, 1.000000000000000000 ) ) ;
#44379=EDGE_CURVE ( 'NONE', #126922, #2437, #42054, .T. ) ;
#44380=DIRECTION ( 'NONE',  ( -0.000000000000000000, -1.000000000000000000, -0.000000000000000000 ) ) ;
#44381=ORIENTED_EDGE ( 'NONE', *, *, #41872, .F. ) ;
#44382=ORIENTED_EDGE ( 'NONE', *, *, #82819, .F. ) ;
#44383=VERTEX_POINT ( 'NONE', #64255 ) ;
#44384=EDGE_LOOP ( 'NONE', ( #78967, #5686 ) ) ;
#44385=DIRECTION ( 'NONE',  ( 0.000000000000000000, 0.000000000000000000, 1.000000000000000000 ) ) ;
#44386=CIRCLE ( 'NONE', #23458, 0.06509327318403745899 ) ;
#44387=CIRCLE ( 'NONE', #50653, 0.06509327318403741736 ) ;
#44388=ADVANCED_FACE ( 'NONE', ( #41424 ), #24345, .T. ) ;
#44389=PLANE ( 'NONE',  #105242 ) ;
#44390=DIRECTION ( 'NONE',  ( -4.274815082592931898E-19, -0.9999939076577903929, -0.003490651415223739937 ) ) ;
#44391=EDGE_CURVE ( 'NONE', #112116, #66867, #112081, .T. ) ;
#44392=LINE ( 'NONE', #103968, #89545 ) ;
#44393=AXIS2_PLACEMENT_3D ( 'NONE', #34932, #24450, #74841 ) ;
#44394=EDGE_CURVE ( 'NONE', #31481, #16149, #45191, .T. ) ;
#44395=ORIENTED_EDGE ( 'NONE', *, *, #26714, .T. ) ;
#44396=AXIS2_PLACEMENT_3D ( 'NONE', #92848, #43757, #123566 ) ;
#44397=AXIS2_PLACEMENT_3D ( 'NONE', #21632, #123669, #52376 ) ;
#44398=CARTESIAN_POINT ( 'NONE',  ( -8.550000000000009592, 2.500000000000000000, 6.841600689897072485 ) ) ;
#44399=AXIS2_PLACEMENT_3D ( 'NONE', #8707, #127234, #48668 ) ;
#44400=ORIENTED_EDGE ( 'NONE', *, *, #14737, .T. ) ;
#44401=DIRECTION ( 'NONE',  ( 0.000000000000000000, -0.9999939076577903929, 0.003490651415223739937 ) ) ;
#44403=CIRCLE ( 'NONE', #61127, 0.1000000000000002554 ) ;
#44404=LINE ( 'NONE', #111192, #79806 ) ;
#44405=CARTESIAN_POINT ( 'NONE',  ( 18.87984495337918744, -0.5408627091910198637, 4.542689527608487765 ) ) ;
#44406=CIRCLE ( 'NONE', #10926, 0.06509327318403745899 ) ;
#44407=ORIENTED_EDGE ( 'NONE', *, *, #121339, .F. ) ;
#44408=ORIENTED_EDGE ( 'NONE', *, *, #31695, .F. ) ;
#44409=ORIENTED_EDGE ( 'NONE', *, *, #12303, .F. ) ;
#44410=DIRECTION ( 'NONE',  ( 0.000000000000000000, 1.000000000000000000, 0.000000000000000000 ) ) ;
#44411=DIRECTION ( 'NONE',  ( 0.000000000000000000, 0.000000000000000000, -1.000000000000000000 ) ) ;
#44412=DIRECTION ( 'NONE',  ( 0.000000000000000000, 1.000000000000000000, 0.000000000000000000 ) ) ;
#44413=FACE_BOUND ( 'NONE', #41526, .T. ) ;
#44414=DIRECTION ( 'NONE',  ( 0.000000000000000000, 0.000000000000000000, 1.000000000000000000 ) ) ;
#44415=FACE_OUTER_BOUND ( 'NONE', #23402, .T. ) ;
#44416=CARTESIAN_POINT ( 'NONE',  ( -13.09999999999999254, 2.500000000000000000, -0.2464101615137741230 ) ) ;
#44417=CONICAL_SURFACE ( 'NONE', #84119, 0.1000000000000002554, 0.003490658503988666988 ) ;
#44419=DIRECTION ( 'NONE',  ( -0.000000000000000000, 1.000000000000000000, -0.000000000000000000 ) ) ;
#44421=VERTEX_POINT ( 'NONE', #14498 ) ;
#44422=CIRCLE ( 'NONE', #44512, 0.09999999999999982514 ) ;
#44423=CIRCLE ( 'NONE', #86263, 0.06509327318403745899 ) ;
#44424=DIRECTION ( 'NONE',  ( 0.000000000000000000, 1.000000000000000000, 0.000000000000000000 ) ) ;
#44425=EDGE_LOOP ( 'NONE', ( #15608, #20655, #128349, #97427 ) ) ;
#44426=ORIENTED_EDGE ( 'NONE', *, *, #49906, .T. ) ;
#44427=ORIENTED_EDGE ( 'NONE', *, *, #30011, .T. ) ;
#44428=ORIENTED_EDGE ( 'NONE', *, *, #49867, .F. ) ;
#44430=EDGE_CURVE ( 'NONE', #21815, #85672, #13768, .T. ) ;
#44431=FACE_BOUND ( 'NONE', #87675, .T. ) ;
#44432=AXIS2_PLACEMENT_3D ( 'NONE', #44903, #105749, #5588 ) ;
#44433=CARTESIAN_POINT ( 'NONE',  ( -5.400000000000023448, 2.500000000000000000, -5.022947341949754119 ) ) ;
#44434=CONICAL_SURFACE ( 'NONE', #4697, 0.1000000000000000472, 0.003490658503988666988 ) ;
#44435=EDGE_CURVE ( 'NONE', #50468, #31778, #38952, .T. ) ;
#44436=AXIS2_PLACEMENT_3D ( 'NONE', #38863, #80699, #11936 ) ;
#44437=AXIS2_PLACEMENT_3D ( 'NONE', #117426, #67707, #107651 ) ;
#44438=EDGE_CURVE ( 'NONE', #125357, #103547, #36790, .T. ) ;
#44440=ORIENTED_EDGE ( 'NONE', *, *, #129115, .F. ) ;
#44441=CARTESIAN_POINT ( 'NONE',  ( -1.250000000000001110, 12.50000000000000000, -6.495190528383302464 ) ) ;
#44442=CARTESIAN_POINT ( 'NONE',  ( 5.199999999999937117, 2.500000000000000000, -4.776537180435978414 ) ) ;
#44443=ORIENTED_EDGE ( 'NONE', *, *, #96639, .F. ) ;
#44444=AXIS2_PLACEMENT_3D ( 'NONE', #52306, #31392, #73876 ) ;
#44445=DIRECTION ( 'NONE',  ( 0.000000000000000000, 1.000000000000000000, 0.000000000000000000 ) ) ;
#44446=CARTESIAN_POINT ( 'NONE',  ( 5.799999999999933209, 2.500000000000000000, -0.1000000000000023925 ) ) ;
#44447=EDGE_CURVE ( 'NONE', #20499, #49010, #86933, .T. ) ;
#44448=AXIS2_PLACEMENT_3D ( 'NONE', #70675, #30775, #20936 ) ;
#44449=AXIS2_PLACEMENT_3D ( 'NONE', #71340, #113200, #92272 ) ;
#44450=VERTEX_POINT ( 'NONE', #121253 ) ;
#44451=FACE_OUTER_BOUND ( 'NONE', #20298, .T. ) ;
#44452=DIRECTION ( 'NONE',  ( 0.000000000000000000, 1.000000000000000000, 0.000000000000000000 ) ) ;
#44453=CIRCLE ( 'NONE', #42415, 0.1000000000000002554 ) ;
#44454=VERTEX_POINT ( 'NONE', #3408 ) ;
#44456=DIRECTION ( 'NONE',  ( 0.000000000000000000, 0.000000000000000000, 1.000000000000000000 ) ) ;
#44457=DIRECTION ( 'NONE',  ( -0.000000000000000000, -1.000000000000000000, -0.000000000000000000 ) ) ;
#44458=ORIENTED_EDGE ( 'NONE', *, *, #13821, .F. ) ;
#44459=ORIENTED_EDGE ( 'NONE', *, *, #115427, .T. ) ;
#44460=LINE ( 'NONE', #84387, #105800 ) ;
#44461=ADVANCED_FACE ( 'NONE', ( #31588 ), #13213, .T. ) ;
#44462=ORIENTED_EDGE ( 'NONE', *, *, #9782, .T. ) ;
#44463=DIRECTION ( 'NONE',  ( -4.274815082592931898E-19, -0.9999939076577903929, -0.003490651415223739937 ) ) ;
#44464=DIRECTION ( 'NONE',  ( 0.000000000000000000, 1.000000000000000000, 0.000000000000000000 ) ) ;
#44465=EDGE_LOOP ( 'NONE', ( #10052, #84219 ) ) ;
#44466=CARTESIAN_POINT ( 'NONE',  ( -3.750000000000029310, 12.50000000000000000, -7.188010851410854052 ) ) ;
#44467=DIRECTION ( 'NONE',  ( 0.000000000000000000, 1.000000000000000000, 0.000000000000000000 ) ) ;
#44468=CARTESIAN_POINT ( 'NONE',  ( -7.900000000000011013, 2.500000000000000000, 4.330127018922196314 ) ) ;
#44469=DIRECTION ( 'NONE',  ( -0.000000000000000000, 1.000000000000000000, -0.000000000000000000 ) ) ;
#44470=DIRECTION ( 'NONE',  ( -0.000000000000000000, 1.000000000000000000, -0.000000000000000000 ) ) ;
#44471=ORIENTED_EDGE ( 'NONE', *, *, #119329, .F. ) ;
#44472=ORIENTED_EDGE ( 'NONE', *, *, #60242, .F. ) ;
#44473=FACE_OUTER_BOUND ( 'NONE', #46088, .T. ) ;
#44474=ADVANCED_FACE ( 'NONE', ( #122548 ), #124600, .T. ) ;
#44475=CIRCLE ( 'NONE', #92502, 0.06509327318403745899 ) ;
#44477=CIRCLE ( 'NONE', #119689, 0.06509327318403745899 ) ;
#44478=VECTOR ( 'NONE', #123391, 1000.000000000000000 ) ;
#44479=CARTESIAN_POINT ( 'NONE',  ( -1.900000000000034994, 2.500000000000000000, -4.776537180435978414 ) ) ;
#44480=ORIENTED_EDGE ( 'NONE', *, *, #53436, .T. ) ;
#44481=ORIENTED_EDGE ( 'NONE', *, *, #109507, .F. ) ;
#44482=ORIENTED_EDGE ( 'NONE', *, *, #106607, .F. ) ;
#44483=CARTESIAN_POINT ( 'NONE',  ( -0.8500000000000382805, 2.500000000000000000, -5.802370205355749988 ) ) ;
#44484=DIRECTION ( 'NONE',  ( 0.000000000000000000, 0.000000000000000000, 1.000000000000000000 ) ) ;
#44485=VECTOR ( 'NONE', #48399, 1000.000000000000000 ) ;
#44486=LINE ( 'NONE', #113882, #87362 ) ;
#44487=FACE_OUTER_BOUND ( 'NONE', #97991, .T. ) ;
#44488=DIRECTION ( 'NONE',  ( 0.000000000000000000, 1.000000000000000000, 0.000000000000000000 ) ) ;
#44489=CARTESIAN_POINT ( 'NONE',  ( 21.25101288990114412, -0.2446430927199611527, 4.189229928197906183 ) ) ;
#44490=CONICAL_SURFACE ( 'NONE', #48714, 0.1000000000000002554, 0.003490658503988666988 ) ;
#44491=LINE ( 'NONE', #83774, #101455 ) ;
#44492=DIRECTION ( 'NONE',  ( 0.000000000000000000, 1.000000000000000000, 0.000000000000000000 ) ) ;
#44493=AXIS2_PLACEMENT_3D ( 'NONE', #39527, #8720, #29677 ) ;
#44494=EDGE_CURVE ( 'NONE', #108166, #11311, #91148, .T. ) ;
#44495=DIRECTION ( 'NONE',  ( -0.000000000000000000, 1.000000000000000000, -0.000000000000000000 ) ) ;
#44496=AXIS2_PLACEMENT_3D ( 'NONE', #47591, #9591, #78993 ) ;
#44497=ORIENTED_EDGE ( 'NONE', *, *, #39596, .T. ) ;
#44498=DIRECTION ( 'NONE',  ( -4.274815082592931898E-19, -0.9999939076577903929, -0.003490651415223739937 ) ) ;
#44499=ORIENTED_EDGE ( 'NONE', *, *, #71145, .T. ) ;
#44500=ADVANCED_FACE ( 'NONE', ( #43351 ), #101626, .T. ) ;
#44501=VERTEX_POINT ( 'NONE', #83272 ) ;
#44502=DIRECTION ( 'NONE',  ( 0.000000000000000000, 1.000000000000000000, 0.000000000000000000 ) ) ;
#44503=CARTESIAN_POINT ( 'NONE',  ( 9.599999999999917932, 2.500000000000000000, -0.6928203230275541413 ) ) ;
#44504=CARTESIAN_POINT ( 'NONE',  ( -12.29999999999999716, 12.50000000000000000, 0.3464101615137776813 ) ) ;
#44505=AXIS2_PLACEMENT_3D ( 'NONE', #11398, #101727, #40222 ) ;
#44507=DIRECTION ( 'NONE',  ( 0.000000000000000000, 0.000000000000000000, 1.000000000000000000 ) ) ;
#44508=CARTESIAN_POINT ( 'NONE',  ( -12.09999999999999609, 2.500000000000000000, -5.022947341949751454 ) ) ;
#44509=CARTESIAN_POINT ( 'NONE',  ( 9.799999999999915445, 2.500000000000000000, 4.083716857408421497 ) ) ;
#44510=EDGE_LOOP ( 'NONE', ( #69045, #3420, #85709, #22323 ) ) ;
#44511=CARTESIAN_POINT ( 'NONE',  ( -3.550000000000028244, 12.50000000000000000, -1.818653347947326138 ) ) ;
#44512=AXIS2_PLACEMENT_3D ( 'NONE', #13298, #32343, #14586 ) ;
#44513=CARTESIAN_POINT ( 'NONE',  ( 4.599999999999935696, 2.500000000000000000, 5.022947341949748790 ) ) ;
#44514=CONICAL_SURFACE ( 'NONE', #67474, 0.1000000000000000056, 0.003490658503988666988 ) ;
#44515=ORIENTED_EDGE ( 'NONE', *, *, #114546, .T. ) ;
#44516=AXIS2_PLACEMENT_3D ( 'NONE', #48476, #10, #98209 ) ;
#44518=EDGE_CURVE ( 'NONE', #57241, #31023, #23054, .T. ) ;
#44519=ORIENTED_EDGE ( 'NONE', *, *, #110981, .F. ) ;
#44520=ORIENTED_EDGE ( 'NONE', *, *, #106521, .F. ) ;
#44521=CIRCLE ( 'NONE', #105153, 0.1000000000000000472 ) ;
#44522=DIRECTION ( 'NONE',  ( -0.000000000000000000, 1.000000000000000000, -0.000000000000000000 ) ) ;
#44523=CARTESIAN_POINT ( 'NONE',  ( -6.900000000000019007, 2.500000000000000000, -4.676537180435978769 ) ) ;
#44524=CONICAL_SURFACE ( 'NONE', #117656, 0.1000000000000002554, 0.003490658503988666988 ) ;
#44525=AXIS2_PLACEMENT_3D ( 'NONE', #89066, #90323, #59627 ) ;
#44526=EDGE_CURVE ( 'NONE', #47712, #95333, #32891, .T. ) ;
#44527=DIRECTION ( 'NONE',  ( 0.000000000000000000, 0.000000000000000000, 1.000000000000000000 ) ) ;
#44528=AXIS2_PLACEMENT_3D ( 'NONE', #55813, #36829, #96359 ) ;
#44529=DIRECTION ( 'NONE',  ( 0.000000000000000000, 0.000000000000000000, 1.000000000000000000 ) ) ;
#44530=FACE_OUTER_BOUND ( 'NONE', #46599, .T. ) ;
#44531=EDGE_LOOP ( 'NONE', ( #128185, #30799 ) ) ;
#44532=DIRECTION ( 'NONE',  ( 0.000000000000000000, -0.9999939076577903929, 0.003490651415223739937 ) ) ;
#44533=EDGE_CURVE ( 'NONE', #84391, #97166, #57795, .T. ) ;
#44534=EDGE_CURVE ( 'NONE', #24701, #96497, #7605, .T. ) ;
#44535=EDGE_CURVE ( 'NONE', #63642, #12902, #43994, .T. ) ;
#44536=DIRECTION ( 'NONE',  ( -0.000000000000000000, -1.000000000000000000, -0.000000000000000000 ) ) ;
#44537=ADVANCED_FACE ( 'NONE', ( #116571 ), #99574, .T. ) ;
#44538=AXIS2_PLACEMENT_3D ( 'NONE', #125545, #97379, #34622 ) ;
#44539=CARTESIAN_POINT ( 'NONE',  ( -0.2000000000000399791, 2.500000000000000000, -4.676537180435977881 ) ) ;
#44540=ORIENTED_EDGE ( 'NONE', *, *, #82226, .T. ) ;
#44541=VECTOR ( 'NONE', #1829, 1000.000000000000000 ) ;
#44543=VECTOR ( 'NONE', #117057, 1000.000000000000000 ) ;
#44544=VERTEX_POINT ( 'NONE', #16419 ) ;
#44545=EDGE_CURVE ( 'NONE', #117445, #106877, #84970, .T. ) ;
#44546=EDGE_LOOP ( 'NONE', ( #129006, #8555, #111545, #110129 ) ) ;
#44547=CARTESIAN_POINT ( 'NONE',  ( 4.549999999999937650, 12.50000000000000000, 2.165063509461097713 ) ) ;
#44548=EDGE_CURVE ( 'NONE', #88347, #67282, #126755, .T. ) ;
#44549=EDGE_CURVE ( 'NONE', #77475, #113921, #34829, .T. ) ;
#44550=LINE ( 'NONE', #88815, #61357 ) ;
#44551=FACE_OUTER_BOUND ( 'NONE', #48417, .T. ) ;
#44552=EDGE_CURVE ( 'NONE', #125704, #82981, #125737, .T. ) ;
#44553=EDGE_CURVE ( 'NONE', #7894, #82797, #101714, .T. ) ;
#44554=AXIS2_PLACEMENT_3D ( 'NONE', #30630, #69899, #122227 ) ;
#44555=ORIENTED_EDGE ( 'NONE', *, *, #81783, .F. ) ;
#44556=CARTESIAN_POINT ( 'NONE',  ( -9.350000000000004974, 12.50000000000000000, 6.148780366869520897 ) ) ;
#44557=CARTESIAN_POINT ( 'NONE',  ( -14.39999999999998614, 12.50000000000000000, -0.2813168883297386680 ) ) ;
#44558=DIRECTION ( 'NONE',  ( -0.000000000000000000, 1.000000000000000000, -0.000000000000000000 ) ) ;
#44560=FACE_OUTER_BOUND ( 'NONE', #73271, .T. ) ;
#44561=ADVANCED_FACE ( 'NONE', ( #75359 ), #127059, .T. ) ;
#44562=EDGE_LOOP ( 'NONE', ( #106665, #18701 ) ) ;
#44563=DIRECTION ( 'NONE',  ( 0.000000000000000000, 0.000000000000000000, 1.000000000000000000 ) ) ;
#44564=VERTEX_POINT ( 'NONE', #37393 ) ;
#44565=CIRCLE ( 'NONE', #69602, 0.06509327318403741736 ) ;
#44566=ORIENTED_EDGE ( 'NONE', *, *, #32112, .F. ) ;
#44567=AXIS2_PLACEMENT_3D ( 'NONE', #99220, #8876, #48178 ) ;
#44568=CARTESIAN_POINT ( 'NONE',  ( -5.850000000000021849, 2.500000000000000000, -5.702370205355749455 ) ) ;
#44569=CARTESIAN_POINT ( 'NONE',  ( -13.54999999999999005, 2.500000000000000000, -1.718653347947323828 ) ) ;
#44570=DIRECTION ( 'NONE',  ( -0.000000000000000000, 1.000000000000000000, -0.000000000000000000 ) ) ;
#44571=DIRECTION ( 'NONE',  ( 0.000000000000000000, -0.9999939076577903929, 0.003490651415223739937 ) ) ;
#44572=CARTESIAN_POINT ( 'NONE',  ( 11.69999999999990870, 2.500000000000000000, 4.430127018922196847 ) ) ;
#44573=ORIENTED_EDGE ( 'NONE', *, *, #116215, .F. ) ;
#44574=CONICAL_SURFACE ( 'NONE', #52898, 0.1000000000000000472, 0.003490658503988666988 ) ;
#44575=AXIS2_PLACEMENT_3D ( 'NONE', #10345, #117696, #58809 ) ;
#44576=CIRCLE ( 'NONE', #21589, 0.06509327318403745899 ) ;
#44577=ORIENTED_EDGE ( 'NONE', *, *, #98487, .T. ) ;
#44578=CARTESIAN_POINT ( 'NONE',  ( -11.05000000000000071, 2.500000000000000000, -2.511473670974873951 ) ) ;
#44579=DIRECTION ( 'NONE',  ( 0.000000000000000000, 1.000000000000000000, 0.000000000000000000 ) ) ;
#44580=CARTESIAN_POINT ( 'NONE',  ( -11.84999999999999609, 12.50000000000000000, 2.576566944158910744 ) ) ;
#44581=CARTESIAN_POINT ( 'NONE',  ( -6.650000000000018119, 12.50000000000000000, -6.430097255199264339 ) ) ;
#44582=ORIENTED_EDGE ( 'NONE', *, *, #64602, .F. ) ;
#44583=AXIS2_PLACEMENT_3D ( 'NONE', #39419, #40043, #89776 ) ;
#44584=DIRECTION ( 'NONE',  ( -0.000000000000000000, -1.000000000000000000, -0.000000000000000000 ) ) ;
#44585=AXIS2_PLACEMENT_3D ( 'NONE', #98446, #17962, #57910 ) ;
#44586=CARTESIAN_POINT ( 'NONE',  ( 7.099999999999928590, 2.500000000000000000, -5.022947341949754119 ) ) ;
#44587=EDGE_LOOP ( 'NONE', ( #79892, #18899, #98009, #79391 ) ) ;
#44588=AXIS2_PLACEMENT_3D ( 'NONE', #106174, #6633, #107455 ) ;
#44589=DIRECTION ( 'NONE',  ( 0.000000000000000000, 0.000000000000000000, 1.000000000000000000 ) ) ;
#44590=ORIENTED_EDGE ( 'NONE', *, *, #29024, .F. ) ;
#44591=DIRECTION ( 'NONE',  ( 0.000000000000000000, 1.000000000000000000, 0.000000000000000000 ) ) ;
#44592=EDGE_CURVE ( 'NONE', #92201, #71646, #105911, .T. ) ;
#44593=ORIENTED_EDGE ( 'NONE', *, *, #86452, .T. ) ;
#44594=CARTESIAN_POINT ( 'NONE',  ( -5.850000000000018296, 12.50000000000000000, 5.737276932171707422 ) ) ;
#44595=DIRECTION ( 'NONE',  ( 0.000000000000000000, 0.000000000000000000, 1.000000000000000000 ) ) ;
#44596=EDGE_CURVE ( 'NONE', #109510, #54407, #107406, .T. ) ;
#44597=ORIENTED_EDGE ( 'NONE', *, *, #113243, .T. ) ;
#44598=EDGE_LOOP ( 'NONE', ( #98000, #48456, #127765, #101581 ) ) ;
#44600=CONICAL_SURFACE ( 'NONE', #128246, 0.09999999999999982514, 0.003490658503988666988 ) ;
#44601=DIRECTION ( 'NONE',  ( 0.000000000000000000, 1.000000000000000000, 0.000000000000000000 ) ) ;
#44602=DIRECTION ( 'NONE',  ( 0.000000000000000000, 0.000000000000000000, 1.000000000000000000 ) ) ;
#44603=EDGE_CURVE ( 'NONE', #9421, #81291, #15136, .T. ) ;
#44604=CARTESIAN_POINT ( 'NONE',  ( -7.900000000000014566, 2.500000000000000000, -0.5928203230275541635 ) ) ;
#44605=DIRECTION ( 'NONE',  ( 0.000000000000000000, 0.000000000000000000, -1.000000000000000000 ) ) ;
#44606=CARTESIAN_POINT ( 'NONE',  ( -9.800000000000006040, 12.50000000000000000, -4.676537180435974328 ) ) ;
#44607=DIRECTION ( 'NONE',  ( 0.000000000000000000, 0.000000000000000000, 1.000000000000000000 ) ) ;
#44608=AXIS2_PLACEMENT_3D ( 'NONE', #25378, #74499, #103321 ) ;
#44609=CIRCLE ( 'NONE', #59208, 0.09999999999999999167 ) ;
#44610=CONICAL_SURFACE ( 'NONE', #109453, 0.1000000000000002554, 0.003490658503988666988 ) ;
#44611=ORIENTED_EDGE ( 'NONE', *, *, #56966, .F. ) ;
#44612=ORIENTED_EDGE ( 'NONE', *, *, #32226, .T. ) ;
#44613=CARTESIAN_POINT ( 'NONE',  ( 6.899999999999926636, 2.500000000000000000, -0.3464101615137782364 ) ) ;
#44614=CARTESIAN_POINT ( 'NONE',  ( 10.64999999999990976, 2.500000000000000000, 1.718653347947321386 ) ) ;
#44615=CARTESIAN_POINT ( 'NONE',  ( 0.8499999999999536815, 2.500000000000000000, 5.702370205355745014 ) ) ;
#44616=CARTESIAN_POINT ( 'NONE',  ( 14.34999999999989306, 2.500000000000000000, -1.818653347947326138 ) ) ;
#44617=EDGE_LOOP ( 'NONE', ( #96574, #75434, #41955, #51826 ) ) ;
#44618=ORIENTED_EDGE ( 'NONE', *, *, #39649, .T. ) ;
#44619=DIRECTION ( 'NONE',  ( 0.000000000000000000, 0.000000000000000000, -1.000000000000000000 ) ) ;
#44620=ORIENTED_EDGE ( 'NONE', *, *, #2856, .F. ) ;
#44621=FACE_OUTER_BOUND ( 'NONE', #105196, .T. ) ;
#44622=CARTESIAN_POINT ( 'NONE',  ( 4.599999999999939249, 2.500000000000000000, -3.637306695894650055 ) ) ;
#44623=VERTEX_POINT ( 'NONE', #66186 ) ;
#44624=CONICAL_SURFACE ( 'NONE', #15353, 0.1000000000000002554, 0.003490658503988666988 ) ;
#44625=DIRECTION ( 'NONE',  ( 0.000000000000000000, 0.000000000000000000, 1.000000000000000000 ) ) ;
#44626=DIRECTION ( 'NONE',  ( -4.274815082592931898E-19, -0.9999939076577903929, -0.003490651415223739937 ) ) ;
#44627=CONICAL_SURFACE ( 'NONE', #57137, 0.1000000000000002554, 0.003490658503988666988 ) ;
#44628=CARTESIAN_POINT ( 'NONE',  ( -8.100000000000013856, 2.500000000000000000, -4.676537180435977881 ) ) ;
#44629=CARTESIAN_POINT ( 'NONE',  ( 11.84999999999990372, 2.500000000000000000, 2.511473670974873507 ) ) ;
#44630=LINE ( 'NONE', #26285, #85034 ) ;
#44631=DIRECTION ( 'NONE',  ( 0.000000000000000000, 0.000000000000000000, 1.000000000000000000 ) ) ;
#44632=CARTESIAN_POINT ( 'NONE',  ( 12.29999999999990479, 2.500000000000000000, -4.083716857408426826 ) ) ;
#44633=FACE_OUTER_BOUND ( 'NONE', #57446, .T. ) ;
#44634=CIRCLE ( 'NONE', #84339, 0.09999999999999982514 ) ;
#44635=CARTESIAN_POINT ( 'NONE',  ( 3.349999999999943689, 2.500000000000000000, 1.472243186433545459 ) ) ;
#44636=EDGE_CURVE ( 'NONE', #36792, #98705, #4667, .T. ) ;
#44637=ORIENTED_EDGE ( 'NONE', *, *, #39944, .T. ) ;
#44638=VERTEX_POINT ( 'NONE', #114642 ) ;
#44640=CARTESIAN_POINT ( 'NONE',  ( 2.499999999999947153, 2.500000000000000000, -3.637306695894650055 ) ) ;
#44641=CONICAL_SURFACE ( 'NONE', #82203, 0.09999999999999982514, 0.003490658503988666988 ) ;
#44642=EDGE_LOOP ( 'NONE', ( #94963, #63663, #101066, #79580 ) ) ;
#44643=AXIS2_PLACEMENT_3D ( 'NONE', #95873, #44846, #5540 ) ;
#44644=CONICAL_SURFACE ( 'NONE', #84346, 0.09999999999999982514, 0.003490658503988666988 ) ;
#44645=DIRECTION ( 'NONE',  ( 0.000000000000000000, 1.000000000000000000, 0.000000000000000000 ) ) ;
#44646=ORIENTED_EDGE ( 'NONE', *, *, #104659, .F. ) ;
#44647=ORIENTED_EDGE ( 'NONE', *, *, #44548, .F. ) ;
#44648=ORIENTED_EDGE ( 'NONE', *, *, #99079, .F. ) ;
#44649=AXIS2_PLACEMENT_3D ( 'NONE', #40933, #12713, #31106 ) ;
#44650=ADVANCED_FACE ( 'NONE', ( #64893 ), #96935, .T. ) ;
#44651=DIRECTION ( 'NONE',  ( 0.000000000000000000, 0.000000000000000000, -1.000000000000000000 ) ) ;
#44652=CIRCLE ( 'NONE', #11273, 0.06509327318403745899 ) ;
#44653=CARTESIAN_POINT ( 'NONE',  ( 11.84999999999990372, 2.500000000000000000, -6.941600689897078347 ) ) ;
#44654=DIRECTION ( 'NONE',  ( 0.000000000000000000, 0.000000000000000000, 1.000000000000000000 ) ) ;
#44655=CARTESIAN_POINT ( 'NONE',  ( -12.49999999999999289, 2.500000000000000000, 5.122947341949749323 ) ) ;
#44656=ADVANCED_FACE ( 'NONE', ( #95020 ), #89180, .T. ) ;
#44657=CARTESIAN_POINT ( 'NONE',  ( -11.69999999999999929, 12.50000000000000000, 1.734723475976807094E-15 ) ) ;
#44658=VERTEX_POINT ( 'NONE', #45926 ) ;
#44659=FACE_OUTER_BOUND ( 'NONE', #72700, .T. ) ;
#44660=ORIENTED_EDGE ( 'NONE', *, *, #116543, .F. ) ;
#44661=VERTEX_POINT ( 'NONE', #36099 ) ;
#44662=ORIENTED_EDGE ( 'NONE', *, *, #84342, .T. ) ;
#44663=CARTESIAN_POINT ( 'NONE',  ( 10.64999999999991331, 2.500000000000000000, 6.841600689897072485 ) ) ;
#44664=VECTOR ( 'NONE', #16928, 1000.000000000000000 ) ;
#44665=VECTOR ( 'NONE', #39814, 1000.000000000000000 ) ;
#44666=EDGE_LOOP ( 'NONE', ( #123151, #78634 ) ) ;
#44667=EDGE_CURVE ( 'NONE', #77344, #68306, #76012, .T. ) ;
#44668=VERTEX_POINT ( 'NONE', #106120 ) ;
#44669=ORIENTED_EDGE ( 'NONE', *, *, #45921, .T. ) ;
#44670=LINE ( 'NONE', #92470, #31923 ) ;
#44671=VECTOR ( 'NONE', #34927, 1000.000000000000000 ) ;
#44672=DIRECTION ( 'NONE',  ( 0.000000000000000000, 0.000000000000000000, 1.000000000000000000 ) ) ;
#44673=AXIS2_PLACEMENT_3D ( 'NONE', #13597, #73810, #64640 ) ;
#44674=CARTESIAN_POINT ( 'NONE',  ( -6.850000000000013856, 2.500000000000000000, 2.411473670974873862 ) ) ;
#44675=CONICAL_SURFACE ( 'NONE', #92691, 0.1000000000000002554, 0.003490658503988666988 ) ;
#44676=DIRECTION ( 'NONE',  ( 0.000000000000000000, 1.000000000000000000, 0.000000000000000000 ) ) ;
#44677=FACE_OUTER_BOUND ( 'NONE', #93386, .T. ) ;
#44678=AXIS2_PLACEMENT_3D ( 'NONE', #50138, #47552, #109018 ) ;
#44679=AXIS2_PLACEMENT_3D ( 'NONE', #50640, #895, #80757 ) ;
#44680=ORIENTED_EDGE ( 'NONE', *, *, #58774, .F. ) ;
#44681=CARTESIAN_POINT ( 'NONE',  ( 10.59999999999990905, 2.500000000000000000, 4.776537180435972196 ) ) ;
#44682=AXIS2_PLACEMENT_3D ( 'NONE', #4067, #3430, #112753 ) ;
#44683=ORIENTED_EDGE ( 'NONE', *, *, #55364, .T. ) ;
#44684=DIRECTION ( 'NONE',  ( 0.000000000000000000, 0.000000000000000000, 1.000000000000000000 ) ) ;
#44685=AXIS2_PLACEMENT_3D ( 'NONE', #46688, #114772, #74864 ) ;
#44686=ORIENTED_EDGE ( 'NONE', *, *, #81778, .F. ) ;
#44687=FACE_OUTER_BOUND ( 'NONE', #68907, .T. ) ;
#44688=ORIENTED_EDGE ( 'NONE', *, *, #111340, .T. ) ;
#44689=CONICAL_SURFACE ( 'NONE', #57202, 0.1000000000000002554, 0.003490658503988666988 ) ;
#44690=ORIENTED_EDGE ( 'NONE', *, *, #7085, .F. ) ;
#44691=DIRECTION ( 'NONE',  ( 0.000000000000000000, -0.9999939076577903929, 0.003490651415223739937 ) ) ;
#44692=DIRECTION ( 'NONE',  ( 0.000000000000000000, 1.000000000000000000, 0.000000000000000000 ) ) ;
#44693=ADVANCED_FACE ( 'NONE', ( #56367 ), #101508, .T. ) ;
#44694=DIRECTION ( 'NONE',  ( 0.000000000000000000, 0.000000000000000000, -1.000000000000000000 ) ) ;
#44695=ORIENTED_EDGE ( 'NONE', *, *, #61142, .F. ) ;
#44696=DIRECTION ( 'NONE',  ( -0.000000000000000000, 1.000000000000000000, -0.000000000000000000 ) ) ;
#44697=ORIENTED_EDGE ( 'NONE', *, *, #128910, .T. ) ;
#44698=CARTESIAN_POINT ( 'NONE',  ( 9.349999999999916156, 12.50000000000000000, 6.148780366869520009 ) ) ;
#44699=DIRECTION ( 'NONE',  ( -0.000000000000000000, -1.000000000000000000, -0.000000000000000000 ) ) ;
#44701=ADVANCED_FACE ( 'NONE', ( #669 ), #128925, .T. ) ;
#44702=DIRECTION ( 'NONE',  ( 0.000000000000000000, 1.000000000000000000, 0.000000000000000000 ) ) ;
#44703=CARTESIAN_POINT ( 'NONE',  ( 13.14999999999990088, 2.500000000000000000, 2.611473670974873151 ) ) ;
#44704=ADVANCED_FACE ( 'NONE', ( #8539 ), #48488, .T. ) ;
#44705=VECTOR ( 'NONE', #62924, 1000.000000000000000 ) ;
#44706=DIRECTION ( 'NONE',  ( 0.000000000000000000, 0.000000000000000000, 1.000000000000000000 ) ) ;
#44707=ORIENTED_EDGE ( 'NONE', *, *, #57727, .T. ) ;
#44708=ORIENTED_EDGE ( 'NONE', *, *, #89209, .T. ) ;
#44709=EDGE_CURVE ( 'NONE', #10341, #114322, #95447, .T. ) ;
#44710=EDGE_CURVE ( 'NONE', #89261, #118121, #1348, .T. ) ;
#44711=EDGE_CURVE ( 'NONE', #91607, #75694, #28206, .T. ) ;
#44712=CONICAL_SURFACE ( 'NONE', #46766, 0.1000000000000002554, 0.003490658503988666988 ) ;
#44713=ORIENTED_EDGE ( 'NONE', *, *, #65849, .T. ) ;
#44714=AXIS2_PLACEMENT_3D ( 'NONE', #123169, #25588, #45898 ) ;
#44716=CARTESIAN_POINT ( 'NONE',  ( -8.350000000000013856, 2.500000000000000000, -7.188010851410848723 ) ) ;
#44717=AXIS2_PLACEMENT_3D ( 'NONE', #67753, #67076, #49420 ) ;
#44719=B_SPLINE_CURVE_WITH_KNOTS ( 'NONE', 3,
 ( #55640, #54988, #5241, #45188 ),
 .UNSPECIFIED., .F., .F.,
 ( 4, 4 ),
 ( 0.002015733555955073232, 0.002984807578930272990 ),
 .UNSPECIFIED. ) ;
#44721=DIRECTION ( 'NONE',  ( -4.274815082592931898E-19, -0.9999939076577903929, -0.003490651415223739937 ) ) ;
#44722=CARTESIAN_POINT ( 'NONE',  ( 15.39999999999989022, 2.500000000000000000, 0.09999999999999761857 ) ) ;
#44723=LINE ( 'NONE', #96368, #125578 ) ;
#44724=AXIS2_PLACEMENT_3D ( 'NONE', #38496, #99333, #67924 ) ;
#44725=FACE_OUTER_BOUND ( 'NONE', #55503, .T. ) ;
#44726=CIRCLE ( 'NONE', #19582, 0.06509327318403745899 ) ;
#44727=EDGE_LOOP ( 'NONE', ( #17263, #7756, #36937, #123371 ) ) ;
#44728=EDGE_CURVE ( 'NONE', #10571, #49210, #32779, .T. ) ;
#44729=AXIS2_PLACEMENT_3D ( 'NONE', #60598, #80870, #90676 ) ;
#44730=CONICAL_SURFACE ( 'NONE', #117856, 0.09999999999999982514, 0.003490658503988666988 ) ;
#44731=DIRECTION ( 'NONE',  ( -4.274815082592931898E-19, -0.9999939076577903929, -0.003490651415223739937 ) ) ;
#44732=CARTESIAN_POINT ( 'NONE',  ( 2.899999999999946620, 2.500000000000000000, 0.6928203230275494784 ) ) ;
#44733=ORIENTED_EDGE ( 'NONE', *, *, #80516, .T. ) ;
#44734=AXIS2_PLACEMENT_3D ( 'NONE', #37072, #95337, #67127 ) ;
#44735=DIRECTION ( 'NONE',  ( 0.000000000000000000, 0.000000000000000000, 1.000000000000000000 ) ) ;
#44736=ORIENTED_EDGE ( 'NONE', *, *, #41797, .F. ) ;
#44737=AXIS2_PLACEMENT_3D ( 'NONE', #57125, #64997, #55838 ) ;
#44738=AXIS2_PLACEMENT_3D ( 'NONE', #101023, #31024, #62403 ) ;
#44739=CONICAL_SURFACE ( 'NONE', #55197, 0.09999999999999999167, 0.003490658503988666988 ) ;
#44740=CARTESIAN_POINT ( 'NONE',  ( -8.150000000000009237, 2.500000000000000000, 6.841600689897072485 ) ) ;
#44741=VECTOR ( 'NONE', #96429, 1000.000000000000000 ) ;
#44742=ORIENTED_EDGE ( 'NONE', *, *, #102682, .T. ) ;
#44743=DIRECTION ( 'NONE',  ( -0.000000000000000000, 1.000000000000000000, -0.000000000000000000 ) ) ;
#44744=DIRECTION ( 'NONE',  ( 0.000000000000000000, 0.000000000000000000, 1.000000000000000000 ) ) ;
#44745=CARTESIAN_POINT ( 'NONE',  ( 1.249999999999986899, 2.500000000000000000, 6.595190528383296780 ) ) ;
#44746=CIRCLE ( 'NONE', #61480, 0.1000000000000000472 ) ;
#44747=ORIENTED_EDGE ( 'NONE', *, *, #103053, .T. ) ;
#44749=PLANE ( 'NONE',  #26564 ) ;
#44750=EDGE_LOOP ( 'NONE', ( #63325, #123806, #29221, #82616 ) ) ;
#44751=DIRECTION ( 'NONE',  ( 0.000000000000000000, -0.000000000000000000, 1.000000000000000000 ) ) ;
#44752=ADVANCED_FACE ( 'NONE', ( #89062 ), #59625, .T. ) ;
#44753=EDGE_LOOP ( 'NONE', ( #128439, #95386, #39981, #33645 ) ) ;
#44754=ORIENTED_EDGE ( 'NONE', *, *, #37209, .T. ) ;
#44755=DIRECTION ( 'NONE',  ( 0.000000000000000000, 0.000000000000000000, -1.000000000000000000 ) ) ;
#44756=CARTESIAN_POINT ( 'NONE',  ( -11.05000000000000071, 2.500000000000000000, 2.611473670974873151 ) ) ;
#44757=VECTOR ( 'NONE', #124534, 1000.000000000000000 ) ;
#44758=CIRCLE ( 'NONE', #128295, 0.06509327318403745899 ) ;
#44759=AXIS2_PLACEMENT_3D ( 'NONE', #78452, #118346, #117036 ) ;
#44760=ORIENTED_EDGE ( 'NONE', *, *, #96587, .F. ) ;
#44761=CARTESIAN_POINT ( 'NONE',  ( 12.49999999999993605, 2.500000000000000000, -2.276824562219559311E-15 ) ) ;
#44762=CARTESIAN_POINT ( 'NONE',  ( 6.649999999999928413, 12.50000000000000000, 1.472243186433545459 ) ) ;
#44763=EDGE_LOOP ( 'NONE', ( #1128, #65971, #46773, #22802 ) ) ;
#44764=ADVANCED_FACE ( 'NONE', ( #99536 ), #87030, .T. ) ;
#44765=DIRECTION ( 'NONE',  ( 0.000000000000000000, 1.000000000000000000, 0.000000000000000000 ) ) ;
#44766=DIRECTION ( 'NONE',  ( 0.000000000000000000, 1.000000000000000000, 0.000000000000000000 ) ) ;
#44767=AXIS2_PLACEMENT_3D ( 'NONE', #49531, #29250, #119531 ) ;
#44768=AXIS2_PLACEMENT_3D ( 'NONE', #80359, #120279, #129478 ) ;
#44769=VECTOR ( 'NONE', #57704, 1000.000000000000000 ) ;
#44770=CARTESIAN_POINT ( 'NONE',  ( 3.349999999999943689, 12.50000000000000000, 2.165063509461097713 ) ) ;
#44771=DIRECTION ( 'NONE',  ( 0.000000000000000000, 0.000000000000000000, 1.000000000000000000 ) ) ;
#44772=DIRECTION ( 'NONE',  ( 0.000000000000000000, -0.9999939076577903929, 0.003490651415223739937 ) ) ;
#44773=CARTESIAN_POINT ( 'NONE',  ( -12.29999999999999538, 2.500000000000000000, -4.776537180435975749 ) ) ;
#44775=AXIS2_PLACEMENT_3D ( 'NONE', #49724, #89627, #39902 ) ;
#44776=CIRCLE ( 'NONE', #88590, 0.06509327318403745899 ) ;
#44778=ORIENTED_EDGE ( 'NONE', *, *, #88566, .T. ) ;
#44779=ORIENTED_EDGE ( 'NONE', *, *, #117960, .T. ) ;
#44780=ORIENTED_EDGE ( 'NONE', *, *, #62853, .F. ) ;
#44781=ORIENTED_EDGE ( 'NONE', *, *, #50314, .F. ) ;
#44782=FACE_OUTER_BOUND ( 'NONE', #108017, .T. ) ;
#44783=CARTESIAN_POINT ( 'NONE',  ( -6.850000000000017408, 2.500000000000000000, -6.148780366869526226 ) ) ;
#44784=CONICAL_SURFACE ( 'NONE', #113740, 0.09999999999999982514, 0.003490658503988666988 ) ;
#44785=DIRECTION ( 'NONE',  ( -4.274815082592931898E-19, -0.9999939076577903929, -0.003490651415223739937 ) ) ;
#44786=EDGE_LOOP ( 'NONE', ( #118217, #97615 ) ) ;
#44787=FACE_BOUND ( 'NONE', #75524, .T. ) ;
#44788=CARTESIAN_POINT ( 'NONE',  ( 3.949999999999940670, 2.500000000000000000, 1.818653347947321475 ) ) ;
#44789=CARTESIAN_POINT ( 'NONE',  ( -0.8500000000000382805, 2.500000000000000000, -7.088010851410853519 ) ) ;
#44790=CARTESIAN_POINT ( 'NONE',  ( -5.650000000000019895, 12.50000000000000000, 2.446380397790835826 ) ) ;
#44791=DIRECTION ( 'NONE',  ( -4.274815082592931898E-19, -0.9999939076577903929, -0.003490651415223739937 ) ) ;
#44792=DIRECTION ( 'NONE',  ( 0.000000000000000000, 0.000000000000000000, 1.000000000000000000 ) ) ;
#44793=CIRCLE ( 'NONE', #117928, 0.06509327318403745899 ) ;
#44794=DIRECTION ( 'NONE',  ( 0.000000000000000000, 0.000000000000000000, 1.000000000000000000 ) ) ;
#44795=DIRECTION ( 'NONE',  ( 0.000000000000000000, 0.000000000000000000, -1.000000000000000000 ) ) ;
#44796=DIRECTION ( 'NONE',  ( -0.000000000000000000, -1.000000000000000000, -0.000000000000000000 ) ) ;
#44797=CARTESIAN_POINT ( 'NONE',  ( -6.650000000000015454, 12.50000000000000000, 7.253104124594885960 ) ) ;
#44798=AXIS2_PLACEMENT_3D ( 'NONE', #109952, #9163, #40587 ) ;
#44799=LINE ( 'NONE', #104971, #79489 ) ;
#44800=EDGE_CURVE ( 'NONE', #114066, #72352, #59878, .T. ) ;
#44801=EDGE_LOOP ( 'NONE', ( #114424, #4206 ) ) ;
#44802=ORIENTED_EDGE ( 'NONE', *, *, #69329, .T. ) ;
#44803=ORIENTED_EDGE ( 'NONE', *, *, #63, .T. ) ;
#44804=EDGE_LOOP ( 'NONE', ( #68052, #78239 ) ) ;
#44805=FACE_OUTER_BOUND ( 'NONE', #7878, .T. ) ;
#44806=ORIENTED_EDGE ( 'NONE', *, *, #59039, .T. ) ;
#44807=PLANE ( 'NONE',  #46446 ) ;
#44808=VERTEX_POINT ( 'NONE', #2587 ) ;
#44809=ORIENTED_EDGE ( 'NONE', *, *, #24167, .T. ) ;
#44810=AXIS2_PLACEMENT_3D ( 'NONE', #128839, #70521, #126390 ) ;
#44811=EDGE_CURVE ( 'NONE', #75790, #79023, #123037, .T. ) ;
#44812=AXIS2_PLACEMENT_3D ( 'NONE', #117156, #127647, #116531 ) ;
#44813=CARTESIAN_POINT ( 'NONE',  ( 2.500000000000002220, -1.499999999999999556, 10.00000000000000178 ) ) ;
#44814=CARTESIAN_POINT ( 'NONE',  ( 5.599999999999933031, 12.50000000000000000, 0.3464101615137735735 ) ) ;
#44815=LINE ( 'NONE', #54602, #11248 ) ;
#44816=DIRECTION ( 'NONE',  ( 0.000000000000000000, 1.000000000000000000, 0.000000000000000000 ) ) ;
#44817=EDGE_CURVE ( 'NONE', #88216, #68655, #105817, .T. ) ;
#44818=ADVANCED_FACE ( 'NONE', ( #13703 ), #36868, .T. ) ;
#44819=ORIENTED_EDGE ( 'NONE', *, *, #109597, .T. ) ;
#44820=ORIENTED_EDGE ( 'NONE', *, *, #80240, .T. ) ;
#44821=AXIS2_PLACEMENT_3D ( 'NONE', #46818, #40885, #21208 ) ;
#44822=VERTEX_POINT ( 'NONE', #20960 ) ;
#44823=DIRECTION ( 'NONE',  ( 0.000000000000000000, 0.000000000000000000, 1.000000000000000000 ) ) ;
#44824=ORIENTED_EDGE ( 'NONE', *, *, #50079, .F. ) ;
#44825=ADVANCED_FACE ( 'NONE', ( #51719 ), #22906, .T. ) ;
#44827=VERTEX_POINT ( 'NONE', #1949 ) ;
#44828=EDGE_CURVE ( 'NONE', #114539, #126729, #53597, .T. ) ;
#44829=ORIENTED_EDGE ( 'NONE', *, *, #30229, .T. ) ;
#44830=FACE_OUTER_BOUND ( 'NONE', #10060, .T. ) ;
#44831=FACE_OUTER_BOUND ( 'NONE', #3582, .T. ) ;
#44832=AXIS2_PLACEMENT_3D ( 'NONE', #122503, #61656, #91746 ) ;
#44833=CARTESIAN_POINT ( 'NONE',  ( 11.44999999999990514, 2.500000000000000000, 2.411473670974873862 ) ) ;
#44834=AXIS2_PLACEMENT_3D ( 'NONE', #30914, #71452, #22386 ) ;
#44835=DIRECTION ( 'NONE',  ( 0.000000000000000000, 0.000000000000000000, 1.000000000000000000 ) ) ;
#44836=CARTESIAN_POINT ( 'NONE',  ( 15.19999999999989093, 12.50000000000000000, 0.3464101615137735735 ) ) ;
#44837=CIRCLE ( 'NONE', #128464, 0.06509327318403745899 ) ;
#44838=ORIENTED_EDGE ( 'NONE', *, *, #96261, .T. ) ;
#44839=CONICAL_SURFACE ( 'NONE', #46891, 0.1000000000000002554, 0.003490658503988666988 ) ;
#44840=FACE_OUTER_BOUND ( 'NONE', #75180, .T. ) ;
#44841=ORIENTED_EDGE ( 'NONE', *, *, #29178, .T. ) ;
#44842=DIRECTION ( 'NONE',  ( 0.000000000000000000, 0.000000000000000000, 1.000000000000000000 ) ) ;
#44843=ORIENTED_EDGE ( 'NONE', *, *, #110048, .T. ) ;
#44844=CARTESIAN_POINT ( 'NONE',  ( -1.650000000000035660, 2.500000000000000000, 7.088010851410848190 ) ) ;
#44845=CARTESIAN_POINT ( 'NONE',  ( -10.85000000000000142, 12.50000000000000000, -1.472243186433546125 ) ) ;
#44846=DIRECTION ( 'NONE',  ( 0.000000000000000000, 1.000000000000000000, 0.000000000000000000 ) ) ;
#44847=LINE ( 'NONE', #104402, #79123 ) ;
#44848=ORIENTED_EDGE ( 'NONE', *, *, #471, .F. ) ;
#44849=CARTESIAN_POINT ( 'NONE',  ( -8.150000000000012790, 2.500000000000000000, 1.718653347947321386 ) ) ;
#44850=ADVANCED_FACE ( 'NONE', ( #72651 ), #30620, .T. ) ;
#44851=AXIS2_PLACEMENT_3D ( 'NONE', #90372, #715, #72694 ) ;
#44852=AXIS2_PLACEMENT_3D ( 'NONE', #51613, #91529, #72544 ) ;
#44853=DIRECTION ( 'NONE',  ( 0.000000000000000000, 0.000000000000000000, -1.000000000000000000 ) ) ;
#44854=ORIENTED_EDGE ( 'NONE', *, *, #26705, .F. ) ;
#44855=ORIENTED_EDGE ( 'NONE', *, *, #82552, .T. ) ;
#44856=VECTOR ( 'NONE', #61260, 1000.000000000000000 ) ;
#44857=CONICAL_SURFACE ( 'NONE', #23926, 0.09999999999999982514, 0.003490658503988666988 ) ;
#44858=EDGE_LOOP ( 'NONE', ( #111450, #30709 ) ) ;
#44860=CARTESIAN_POINT ( 'NONE',  ( 2.949999999999945111, 2.500000000000000000, 2.165063509461097713 ) ) ;
#44862=CARTESIAN_POINT ( 'NONE',  ( 12.09999999999990550, 2.500000000000000000, -3.637306695894650055 ) ) ;
#44863=EDGE_CURVE ( 'NONE', #35583, #10701, #122394, .T. ) ;
#44864=CIRCLE ( 'NONE', #82520, 0.09999999999999982514 ) ;
#44865=CARTESIAN_POINT ( 'NONE',  ( 2.099999999999950351, 2.500000000000000000, -0.7928203230275542301 ) ) ;
#44866=VECTOR ( 'NONE', #100171, 1000.000000000000000 ) ;
#44867=VECTOR ( 'NONE', #14694, 1000.000000000000000 ) ;
#44868=DIRECTION ( 'NONE',  ( -4.274815082592931898E-19, -0.9999939076577903929, -0.003490651415223739937 ) ) ;
#44869=EDGE_CURVE ( 'NONE', #66198, #74685, #120488, .T. ) ;
#44870=ADVANCED_FACE ( 'NONE', ( #60882 ), #16089, .T. ) ;
#44871=EDGE_CURVE ( 'NONE', #4798, #108744, #91242, .T. ) ;
#44872=VERTEX_POINT ( 'NONE', #103393 ) ;
#44873=VECTOR ( 'NONE', #112465, 1000.000000000000000 ) ;
#44874=DIRECTION ( 'NONE',  ( 0.000000000000000000, 1.000000000000000000, 0.000000000000000000 ) ) ;
#44875=AXIS2_PLACEMENT_3D ( 'NONE', #30136, #70046, #60245 ) ;
#44876=ORIENTED_EDGE ( 'NONE', *, *, #111453, .T. ) ;
#44877=EDGE_CURVE ( 'NONE', #38948, #4566, #85068, .T. ) ;
#44878=CIRCLE ( 'NONE', #49187, 0.1000000000000002554 ) ;
#44879=CARTESIAN_POINT ( 'NONE',  ( 3.949999999999942446, 12.50000000000000000, -6.841600689897078702 ) ) ;
#44880=CARTESIAN_POINT ( 'NONE',  ( 12.09999999999990195, 12.50000000000000000, 0.6277270498435120194 ) ) ;
#44881=DIRECTION ( 'NONE',  ( 0.000000000000000000, 1.000000000000000000, 0.000000000000000000 ) ) ;
#44882=ORIENTED_EDGE ( 'NONE', *, *, #102791, .F. ) ;
#44883=EDGE_CURVE ( 'NONE', #126294, #108784, #1312, .T. ) ;
#44884=EDGE_CURVE ( 'NONE', #114224, #36786, #82934, .T. ) ;
#44885=LINE ( 'NONE', #3652, #128696 ) ;
#44886=CARTESIAN_POINT ( 'NONE',  ( -1.250000000000037526, 2.500000000000000000, -5.802370205355749988 ) ) ;
#44887=VECTOR ( 'NONE', #6117, 1000.000000000000000 ) ;
#44888=ORIENTED_EDGE ( 'NONE', *, *, #119266, .F. ) ;
#44889=DIRECTION ( 'NONE',  ( 0.000000000000000000, 0.000000000000000000, 1.000000000000000000 ) ) ;
#44890=ORIENTED_EDGE ( 'NONE', *, *, #99237, .T. ) ;
#44891=ORIENTED_EDGE ( 'NONE', *, *, #106313, .T. ) ;
#44892=CARTESIAN_POINT ( 'NONE',  ( 7.899999999999924860, 12.50000000000000000, 5.022947341949748790 ) ) ;
#44893=EDGE_LOOP ( 'NONE', ( #10664, #102302, #22153, #10358 ) ) ;
#44894=CARTESIAN_POINT ( 'NONE',  ( 11.89999999999990798, 2.500000000000000000, 4.083716857408421497 ) ) ;
#44896=AXIS2_PLACEMENT_3D ( 'NONE', #101927, #22091, #43664 ) ;
#44897=CARTESIAN_POINT ( 'NONE',  ( -11.89999999999999680, 12.50000000000000000, 0.4115034346978150848 ) ) ;
#44898=VERTEX_POINT ( 'NONE', #121728 ) ;
#44899=FACE_BOUND ( 'NONE', #112626, .T. ) ;
#44900=DIRECTION ( 'NONE',  ( 0.000000000000000000, 0.000000000000000000, 1.000000000000000000 ) ) ;
#44901=DIRECTION ( 'NONE',  ( -0.000000000000000000, 1.000000000000000000, -0.000000000000000000 ) ) ;
#44903=CARTESIAN_POINT ( 'NONE',  ( 13.54999999999990123, 12.50000000000000000, 1.818653347947321475 ) ) ;
#44904=DIRECTION ( 'NONE',  ( -0.000000000000000000, -1.000000000000000000, -0.000000000000000000 ) ) ;
#44905=ORIENTED_EDGE ( 'NONE', *, *, #50795, .F. ) ;
#44906=AXIS2_PLACEMENT_3D ( 'NONE', #32360, #72265, #12665 ) ;
#44907=ORIENTED_EDGE ( 'NONE', *, *, #68361, .T. ) ;
#44908=CIRCLE ( 'NONE', #3050, 0.06509327318403745899 ) ;
#44909=VERTEX_POINT ( 'NONE', #111921 ) ;
#44910=DIRECTION ( 'NONE',  ( 0.000000000000000000, 0.000000000000000000, 1.000000000000000000 ) ) ;
#44911=DIRECTION ( 'NONE',  ( 0.000000000000000000, 0.000000000000000000, 1.000000000000000000 ) ) ;
#44912=DIRECTION ( 'NONE',  ( -4.274815082592931898E-19, -0.9999939076577903929, -0.003490651415223739937 ) ) ;
#44913=FACE_BOUND ( 'NONE', #3202, .T. ) ;
#44914=ORIENTED_EDGE ( 'NONE', *, *, #83399, .F. ) ;
#44916=DIRECTION ( 'NONE',  ( 0.000000000000000000, 0.000000000000000000, -1.000000000000000000 ) ) ;
#44917=CARTESIAN_POINT ( 'NONE',  ( -5.650000000000023448, 12.50000000000000000, -6.148780366869526226 ) ) ;
#44918=ADVANCED_FACE ( 'NONE', ( #23529 ), #118510, .T. ) ;
#44919=DIRECTION ( 'NONE',  ( -0.000000000000000000, -1.000000000000000000, -0.000000000000000000 ) ) ;
#44920=AXIS2_PLACEMENT_3D ( 'NONE', #100473, #103044, #11447 ) ;
#44921=CARTESIAN_POINT ( 'NONE',  ( 9.149999999999915090, 12.50000000000000000, -2.099970236277064473 ) ) ;
#44922=PLANE ( 'NONE',  #52835 ) ;
#44923=AXIS2_PLACEMENT_3D ( 'NONE', #87105, #47850, #108685 ) ;
#44924=CARTESIAN_POINT ( 'NONE',  ( 3.749999999999940492, 12.50000000000000000, 5.802370205355744659 ) ) ;
#44925=VECTOR ( 'NONE', #15424, 1000.000000000000000 ) ;
#44926=LINE ( 'NONE', #63916, #24384 ) ;
#44927=ORIENTED_EDGE ( 'NONE', *, *, #66694, .T. ) ;
#44928=ORIENTED_EDGE ( 'NONE', *, *, #92994, .F. ) ;
#44929=VERTEX_POINT ( 'NONE', #121092 ) ;
#44930=VERTEX_POINT ( 'NONE', #22272 ) ;
#44932=DIRECTION ( 'NONE',  ( 0.000000000000000000, 1.000000000000000000, 0.000000000000000000 ) ) ;
#44933=LINE ( 'NONE', #46208, #111434 ) ;
#44934=VERTEX_POINT ( 'NONE', #21609 ) ;
#44935=FACE_BOUND ( 'NONE', #8859, .T. ) ;
#44936=DIRECTION ( 'NONE',  ( 0.000000000000000000, -0.000000000000000000, 1.000000000000000000 ) ) ;
#44937=AXIS2_PLACEMENT_3D ( 'NONE', #106651, #106016, #98115 ) ;
#44938=FACE_OUTER_BOUND ( 'NONE', #109766, .T. ) ;
#44939=AXIS2_PLACEMENT_3D ( 'NONE', #97961, #19392, #110361 ) ;
#44940=ORIENTED_EDGE ( 'NONE', *, *, #15050, .T. ) ;
#44941=VECTOR ( 'NONE', #6286, 1000.000000000000000 ) ;
#44942=CARTESIAN_POINT ( 'NONE',  ( -2.499999999999996003, 2.500000000000000000, -2.276824562219559311E-15 ) ) ;
#44944=DIRECTION ( 'NONE',  ( -0.000000000000000000, -1.000000000000000000, -0.000000000000000000 ) ) ;
#44945=EDGE_LOOP ( 'NONE', ( #126814, #59824, #28243, #103196 ) ) ;
#44946=DIRECTION ( 'NONE',  ( 0.000000000000000000, 0.000000000000000000, -1.000000000000000000 ) ) ;
#44947=CONICAL_SURFACE ( 'NONE', #78412, 0.1000000000000002554, 0.003490658503988666988 ) ;
#44948=VERTEX_POINT ( 'NONE', #11776 ) ;
#44949=AXIS2_PLACEMENT_3D ( 'NONE', #56206, #45766, #7101 ) ;
#44950=CIRCLE ( 'NONE', #105587, 0.06509327318403745899 ) ;
#44951=VERTEX_POINT ( 'NONE', #7102 ) ;
#44952=ORIENTED_EDGE ( 'NONE', *, *, #23932, .T. ) ;
#44953=FACE_OUTER_BOUND ( 'NONE', #46980, .T. ) ;
#44954=CIRCLE ( 'NONE', #99332, 0.06509327318403745899 ) ;
#44956=DIRECTION ( 'NONE',  ( -0.000000000000000000, -1.000000000000000000, -0.000000000000000000 ) ) ;
#44957=EDGE_LOOP ( 'NONE', ( #38738, #88450, #3576, #59885 ) ) ;
#44958=CARTESIAN_POINT ( 'NONE',  ( 8.497934422428871315, 1.499999999999872768, -9.526046680185359605 ) ) ;
#44959=AXIS2_PLACEMENT_3D ( 'NONE', #13589, #105200, #65917 ) ;
#44960=CONICAL_SURFACE ( 'NONE', #86801, 0.1000000000000002554, 0.003490658503988666988 ) ;
#44961=ADVANCED_FACE ( 'NONE', ( #47054 ), #24828, .T. ) ;
#44962=DIRECTION ( 'NONE',  ( 0.000000000000000000, 0.000000000000000000, 1.000000000000000000 ) ) ;
#44963=LINE ( 'NONE', #104509, #22367 ) ;
#44965=FACE_OUTER_BOUND ( 'NONE', #27111, .T. ) ;
#44966=CIRCLE ( 'NONE', #13638, 0.06509327318403745899 ) ;
#44967=ADVANCED_FACE ( 'NONE', ( #26121 ), #116359, .T. ) ;
#44968=DIRECTION ( 'NONE',  ( 0.000000000000000000, 1.000000000000000000, 0.000000000000000000 ) ) ;
#44969=ADVANCED_FACE ( 'NONE', ( #35305 ), #47429, .T. ) ;
#44970=EDGE_LOOP ( 'NONE', ( #34106, #7239 ) ) ;
#44971=DIRECTION ( 'NONE',  ( -0.000000000000000000, -1.000000000000000000, -0.000000000000000000 ) ) ;
#44972=ORIENTED_EDGE ( 'NONE', *, *, #125476, .F. ) ;
#44973=ORIENTED_EDGE ( 'NONE', *, *, #45778, .F. ) ;
#44974=FACE_OUTER_BOUND ( 'NONE', #43932, .T. ) ;
#44975=DIRECTION ( 'NONE',  ( -0.000000000000000000, -1.000000000000000000, -0.000000000000000000 ) ) ;
#44976=EDGE_CURVE ( 'NONE', #44564, #81764, #62103, .T. ) ;
#44977=EDGE_CURVE ( 'NONE', #56014, #24119, #124783, .T. ) ;
#44978=DIRECTION ( 'NONE',  ( 0.000000000000000000, 1.000000000000000000, 0.000000000000000000 ) ) ;
#44979=DIRECTION ( 'NONE',  ( -0.000000000000000000, -1.000000000000000000, -0.000000000000000000 ) ) ;
#44980=EDGE_CURVE ( 'NONE', #116662, #72184, #1434, .T. ) ;
#44982=CIRCLE ( 'NONE', #28248, 0.06509327318403745899 ) ;
#44983=ORIENTED_EDGE ( 'NONE', *, *, #111642, .T. ) ;
#44984=ORIENTED_EDGE ( 'NONE', *, *, #19260, .F. ) ;
#44986=CARTESIAN_POINT ( 'NONE',  ( -9.350000000000008527, 2.500000000000000000, -6.841600689897072485 ) ) ;
#44987=DIRECTION ( 'NONE',  ( 0.000000000000000000, 0.000000000000000000, 1.000000000000000000 ) ) ;
#44990=DIRECTION ( 'NONE',  ( 0.000000000000000000, 1.000000000000000000, 0.000000000000000000 ) ) ;
#44991=VECTOR ( 'NONE', #16588, 1000.000000000000000 ) ;
#44992=EDGE_LOOP ( 'NONE', ( #19169, #2003 ) ) ;
#44993=DIRECTION ( 'NONE',  ( -4.274815082592931898E-19, -0.9999939076577903929, -0.003490651415223739937 ) ) ;
#44994=AXIS2_PLACEMENT_3D ( 'NONE', #14925, #5762, #56794 ) ;
#44995=DIRECTION ( 'NONE',  ( -0.000000000000000000, -1.000000000000000000, -0.000000000000000000 ) ) ;
#44996=EDGE_LOOP ( 'NONE', ( #92052, #83750, #114012, #80946 ) ) ;
#44997=CARTESIAN_POINT ( 'NONE',  ( 11.84999999999990372, 2.500000000000000000, -6.148780366869526226 ) ) ;
#44998=DIRECTION ( 'NONE',  ( 0.000000000000000000, 1.000000000000000000, 0.000000000000000000 ) ) ;
#44999=FACE_OUTER_BOUND ( 'NONE', #16885, .T. ) ;
#45001=ORIENTED_EDGE ( 'NONE', *, *, #123570, .T. ) ;
#45002=CONICAL_SURFACE ( 'NONE', #118143, 0.1000000000000002554, 0.003490658503988666988 ) ;
#45003=DIRECTION ( 'NONE',  ( -4.274815082592931898E-19, -0.9999939076577903929, -0.003490651415223739937 ) ) ;
#45004=CARTESIAN_POINT ( 'NONE',  ( -10.60000000000000142, 2.500000000000000000, 0.3464101615137736845 ) ) ;
#45005=AXIS2_PLACEMENT_3D ( 'NONE', #93548, #15614, #3872 ) ;
#45006=ORIENTED_EDGE ( 'NONE', *, *, #189, .T. ) ;
#45007=ORIENTED_EDGE ( 'NONE', *, *, #25304, .F. ) ;
#45008=ADVANCED_FACE ( 'NONE', ( #24186 ), #18160, .T. ) ;
#45010=CARTESIAN_POINT ( 'NONE',  ( 3.349999999999943689, 12.50000000000000000, 1.472243186433545459 ) ) ;
#45011=DIRECTION ( 'NONE',  ( -0.000000000000000000, -1.000000000000000000, -0.000000000000000000 ) ) ;
#45012=DIRECTION ( 'NONE',  ( 0.000000000000000000, -0.9999939076577903929, 0.003490651415223739937 ) ) ;
#45013=DIRECTION ( 'NONE',  ( 0.000000000000000000, 0.000000000000000000, -1.000000000000000000 ) ) ;
#45014=AXIS2_PLACEMENT_3D ( 'NONE', #31093, #110272, #110902 ) ;
#45015=CONICAL_SURFACE ( 'NONE', #57624, 0.1000000000000002554, 0.003490658503988666988 ) ;
#45016=DIRECTION ( 'NONE',  ( 0.000000000000000000, -0.9999939076577903929, 0.003490651415223739937 ) ) ;
#45017=CARTESIAN_POINT ( 'NONE',  ( -10.20000000000000284, 2.500000000000000000, -0.3464101615137782364 ) ) ;
#45018=DIRECTION ( 'NONE',  ( 0.000000000000000000, 1.000000000000000000, 0.000000000000000000 ) ) ;
#45019=FACE_OUTER_BOUND ( 'NONE', #112994, .T. ) ;
#45020=EDGE_CURVE ( 'NONE', #71750, #41592, #68343, .T. ) ;
#45021=EDGE_CURVE ( 'NONE', #29207, #109488, #3508, .T. ) ;
#45022=EDGE_CURVE ( 'NONE', #12498, #67302, #101806, .T. ) ;
#45023=FACE_OUTER_BOUND ( 'NONE', #21702, .T. ) ;
#45024=VERTEX_POINT ( 'NONE', #85674 ) ;
#45025=ORIENTED_EDGE ( 'NONE', *, *, #117108, .T. ) ;
#45026=CONICAL_SURFACE ( 'NONE', #84719, 0.09999999999999982514, 0.003490658503988666988 ) ;
#45027=VERTEX_POINT ( 'NONE', #104658 ) ;
#45028=ADVANCED_FACE ( 'NONE', ( #56835 ), #91330, .T. ) ;
#45029=VERTEX_POINT ( 'NONE', #36605 ) ;
#45030=EDGE_CURVE ( 'NONE', #115225, #117649, #72566, .T. ) ;
#45031=CARTESIAN_POINT ( 'NONE',  ( 6.249999999999965361, 12.50000000000000000, 2.165063509461097713 ) ) ;
#45032=AXIS2_PLACEMENT_3D ( 'NONE', #14371, #26151, #54318 ) ;
#45033=DIRECTION ( 'NONE',  ( 0.000000000000000000, 0.000000000000000000, 1.000000000000000000 ) ) ;
#45034=DIRECTION ( 'NONE',  ( 0.000000000000000000, 0.000000000000000000, 1.000000000000000000 ) ) ;
#45035=EDGE_CURVE ( 'NONE', #63269, #87633, #106003, .T. ) ;
#45036=ORIENTED_EDGE ( 'NONE', *, *, #73825, .T. ) ;
#45037=EDGE_CURVE ( 'NONE', #62174, #70962, #66287, .T. ) ;
#45038=DIRECTION ( 'NONE',  ( 0.000000000000000000, 0.000000000000000000, -1.000000000000000000 ) ) ;
#45039=EDGE_CURVE ( 'NONE', #125373, #31532, #124963, .T. ) ;
#45040=CIRCLE ( 'NONE', #15663, 0.1000000000000000472 ) ;
#45041=CARTESIAN_POINT ( 'NONE',  ( -2.950000000000030376, 12.50000000000000000, 6.495190528383297135 ) ) ;
#45042=FACE_OUTER_BOUND ( 'NONE', #2720, .T. ) ;
#45043=VERTEX_POINT ( 'NONE', #126251 ) ;
#45044=CIRCLE ( 'NONE', #95115, 0.06509327318403745899 ) ;
#45045=ADVANCED_FACE ( 'NONE', ( #5809 ), #129015, .T. ) ;
#45046=CARTESIAN_POINT ( 'NONE',  ( 105.5000000000000142, -1.500000000000000222, 1.322875655532295136 ) ) ;
#45047=ORIENTED_EDGE ( 'NONE', *, *, #122922, .T. ) ;
#45048=CONICAL_SURFACE ( 'NONE', #61776, 0.1000000000000002554, 0.003490658503988666988 ) ;
#45049=AXIS2_PLACEMENT_3D ( 'NONE', #85865, #4721, #36153 ) ;
#45050=ORIENTED_EDGE ( 'NONE', *, *, #59486, .F. ) ;
#45051=ORIENTED_EDGE ( 'NONE', *, *, #69665, .F. ) ;
#45052=VERTEX_POINT ( 'NONE', #105965 ) ;
#45054=AXIS2_PLACEMENT_3D ( 'NONE', #82219, #74330, #4921 ) ;
#45055=CARTESIAN_POINT ( 'NONE',  ( 1.849999999999951017, 2.500000000000000000, -6.148780366869526226 ) ) ;
#45056=CARTESIAN_POINT ( 'NONE',  ( 13.34999999999989662, 2.500000000000000000, -2.857883832488653741 ) ) ;
#45057=CIRCLE ( 'NONE', #57577, 0.1000000000000002554 ) ;
#45058=FACE_OUTER_BOUND ( 'NONE', #40614, .T. ) ;
#45059=CIRCLE ( 'NONE', #118200, 0.09999999999999982514 ) ;
#45061=CIRCLE ( 'NONE', #61787, 0.1000000000000000056 ) ;
#45062=DIRECTION ( 'NONE',  ( 0.000000000000000000, 1.000000000000000000, 0.000000000000000000 ) ) ;
#45063=AXIS2_PLACEMENT_3D ( 'NONE', #62889, #13117, #3957 ) ;
#45064=ORIENTED_EDGE ( 'NONE', *, *, #54845, .F. ) ;
#45065=CARTESIAN_POINT ( 'NONE',  ( 35.03103265469133021, -3.271231620378715288, -3.345711933289912121 ) ) ;
#45066=CARTESIAN_POINT ( 'NONE',  ( 2.500000000000002220, -2.499999999999999556, -8.999999999999998224 ) ) ;
#45067=DIRECTION ( 'NONE',  ( -0.000000000000000000, -1.000000000000000000, -0.000000000000000000 ) ) ;
#45068=CARTESIAN_POINT ( 'NONE',  ( 17.34645602450340363, -0.4686430837607939992, 5.377443133677272336 ) ) ;
#45069=EDGE_LOOP ( 'NONE', ( #24995, #4005, #86959, #21130 ) ) ;
#45070=ORIENTED_EDGE ( 'NONE', *, *, #53326, .F. ) ;
#45071=ORIENTED_EDGE ( 'NONE', *, *, #46653, .F. ) ;
#45072=DIRECTION ( 'NONE',  ( -0.000000000000000000, 1.000000000000000000, -0.000000000000000000 ) ) ;
#45074=CARTESIAN_POINT ( 'NONE',  ( -9.600000000000006750, 2.500000000000000000, -0.7928203230275543412 ) ) ;
#45075=FACE_BOUND ( 'NONE', #75119, .T. ) ;
#45076=DIRECTION ( 'NONE',  ( -0.000000000000000000, -1.000000000000000000, -0.000000000000000000 ) ) ;
#45077=AXIS2_PLACEMENT_3D ( 'NONE', #72152, #2095, #74717 ) ;
#45078=DIRECTION ( 'NONE',  ( -0.000000000000000000, -1.000000000000000000, -0.000000000000000000 ) ) ;
#45079=DIRECTION ( 'NONE',  ( -0.000000000000000000, -1.000000000000000000, -0.000000000000000000 ) ) ;
#45080=ADVANCED_FACE ( 'NONE', ( #35935, #16268, #96138, #119004, #129503, #77150, #48334, #39823, #59474, #128191, #37864, #48998, #127542, #28704, #17569, #38542, #117048, #88905, #99377, #78460, #28054, #18215, #67288, #117689, #88225, #57517, #9697, #77773, #49641, #89543, #69244, #118354, #79728, #107248, #37240, #97424, #109167, #7753, #27381, #29355, #18862, #108542, #47699, #87601, #67962, #58173, #107891, #98070, #39186, #8394, #68607, #58804, #98703, #9040, #128857, #79098, #19510, #64517, #104448, #97210, #94619, #124736, #46835, #14749, #6863, #4944, #86073, #37010, #35086, #25896, #5585, #44899, #55984, #54681, #45546, #76929, #17334, #107008, #84804, #85449, #74994, #105078, #116193, #15408, #86740, #127326, #7527, #114902, #95918, #37659, #106380, #96542, #6226, #77557, #25228, #47470, #126675, #126011, #55355, #46173, #36378, #65145, #125384, #95282, #35715, #116834, #76284, #75616, #27177, #115538, #67070, #65805, #26541, #105745, #16049, #66453, #16688, #56617, #57291, #87375, #24607, #127635, #15067, #106064, #104748, #95602, #87057, #67391, #97524, #5904, #16365, #56306, #75948, #16996, #36039, #7850, #127001, #64839, #115880, #47798, #25548, #65485, #106695, #105425, #6528, #94966, #96228, #114580, #56936, #17672, #26861, #86409, #96877, #36697, #107346, #24929, #55023, #57618, #5272, #45220, #87701, #85124, #7200, #125060, #46487, #37341, #35398, #26221, #74669, #75308, #126352, #115204, #45866, #77250, #15735, #55671, #85764, #76606, #116518, #66131, #47151, #117145, #125685, #66770, #27479, #51032, #90939, #68066, #110576, #107991, #50365, #58267, #30753, #89653, #79200, #120406, #90269, #29446, #100119, #109281, #20263, #119745, #108636, #37966, #80493, #18955, #11067, #60836, #611, #89011, #77878, #88331, #78559, #70649, #98812, #59577, #128298, #58905, #118453, #129600, #28804, #10438, #28152, #9152, #117796, #49098, #40577, #69348, #8488, #60212, #18317, #20906, #98169, #99482, #100739, #48432, #39295, #38641, #68710, #19622, #128953, #119108, #9798, #39918, #49742, #79824, #30106, #70017, #109944, #82428, #33330, #103986, #41217, #42499, #14294, #83702, #122346, #81750, #32693, #123604, #53603, #113150, #63414, #73873, #61495, #83064, #71957, #1268, #43794, #111873, #54240, #24138, #13650, #52304, #81128, #51673, #41853, #33957, #62138, #22865, #91582, #72597, #23482, #103348, #121040, #93518, #1903, #52956, #2537, #31389, #64056, #12996, #71283, #3841, #102678, #62779, #102052, #92886, #111202, #21554, #121676, #101410, #113808, #11729, #32040, #22221, #12371, #3214, #112522, #92212, #43156, #122983, #73234, #35886, #76458, #64694, #55532, #104613, #125543, #106548, #56781, #116998, #16849, #15583, #107191, #14916, #5123, #7045, #25396, #115722, #54865, #67236, #4455, #5752, #17516, #47005, #85622, #45075, #126196, #84976, #26071, #36549, #46338, #75794, #84338, #45715, #124912, #65983, #105267, #34619, #35254, #105918, #24782, #75168, #115065, #27329, #126849, #96721, #16216, #94156, #124271, #116365, #44413, #74526, #65327, #95453, #114432, #56153, #94804, #96090, #86908, #37187, #6384, #86252, #26711, #66621, #77101, #99323, #29298, #7697, #97377, #78406, #8986, #30594, #20112, #39140, #128804, #79048, #118307, #118951, #80329, #47644, #107844, #40415, #128137, #50230, #70494, #90116, #28656, #38487, #48284, #9645, #57465, #87549, #58114, #60060, #18813, #58751, #99965, #79671, #88849, #119585, #29939, #127495, #69860, #98018, #109111, #98652, #37816, #120254, #69192, #68556, #108482, #88174, #19458, #59417, #49589, #77721, #445, #117637, #48939, #27997, #89496, #67915, #129452, #10292, #39775, #18168, #109783, #8346, #110418, #13494, #72438, #61975, #103181, #73076, #12207, #82905, #92059, #3056, #120881, #111712, #31234, #52150, #33170, #112998, #11570, #50863, #23314, #102529, #63252, #61330, #53449, #81601, #42331, #71135, #41700, #101246, #112363, #51512, #43004, #123451, #93362, #111039, #2373, #33791, #82262, #122825, #3686, #100589, #43634, #21390, #83552, #91426, #73703, #20754, #60694, #121509, #1742, #31867, #122186, #22705, #32531, #90778, #10899, #41064, #71794, #1106, #22059, #80969, #101895, #62626, #12835, #52786, #92720, #65819, #36391, #46188, #25912, #66467, #4302, #4960, #44913, #45562, #6879, #23983, #34455, #96559, #54701, #106394, #86753, #44246, #16703, #35729, #25241, #56631, #76300, #105095, #86090, #55371, #95936, #84170, #75013, #124101, #15421, #126025, #116207, #104462, #14139, #26555, #105761, #74364, #24626, #46849, #84819, #5596, #114280, #124752, #64536, #14763, #35103, #103829, #94633, #63902, #114916, #126693, #95296, #65160, #6240, #54081, #37022, #113645, #16060, #94002, #85467, #125399, #75632, #115552, #55998, #108954, #78245, #10138, #128650, #48780, #99810, #58601, #77568, #50084, #28492, #19292, #89970, #59905, #59255, #8824, #107694, #98494, #67085, #68399, #67762, #88695, #88018, #17351, #18009, #118150, #7541, #57954, #27832, #290, #109630, #39624, #38987, #99167, #78894, #9493, #76947, #116850, #97862, #108326, #27188, #37672, #118795, #107024, #49432, #89342, #19959, #47486, #29148, #8189, #57306, #119426, #48133, #97224, #87390, #117472, #79525, #38317, #18660, #29771, #129292, #69044, #69696, #127344, #127970, #102387, #40913, #91916, #41548, #40243, #104771, #52002, #120096, #21234, #31087, #111552, #42175, #101740, #110265, #114604, #60549, #11417, #30442, #61168, #80164, #110896, #2897, #71627, #10744, #62475, #15090, #2227, #12058, #21903, #55053, #122028, #112204, #61829, #94983, #90619, #24947, #22550, #82093, #70990, #32385, #72290, #70341, #20604, #12687, #52628, #92555, #42849, #100446, #50698, #82760, #64859, #124440, #34786, #74693, #101090, #1587, #953, #80818, #81460, #120728, #51368, #91271, #121365, #31712, #67414, #5923, #56964, #6550, #35422, #17691, #25573, #127657, #96902, #46507, #87720, #57638, #126374, #107373, #76631, #117165, #105448, #96247, #15754, #36715, #97548, #7873, #125700, #75327, #56325, #18344, #55690, #45885, #47824, #66150, #26882, #95624, #26244, #115222, #106087, #75976, #77271, #65507, #47174, #106714, #85148, #45240, #85787, #37986, #108012, #77900, #116541, #66789, #17013, #16383, #7218, #28174, #125079, #36061, #117819, #115896, #68084, #58287, #5291, #86435, #87076, #127030, #37359, #27497, #89671, #30773, #39939, #80510, #68734, #120423, #48451, #70670, #38661, #30126, #110593, #108657, #99501, #21575, #78581, #44251, #128324, #119133, #20932, #90961, #70037, #121059, #79841, #98834, #31408, #49768, #632, #71307, #8509, #9820, #111217, #51053, #119771, #49118, #40605, #89030, #109963, #118474, #20284, #88356, #28828, #60235, #81149, #100142, #10458, #50386, #79218, #59598, #98193, #18980, #90289, #60855, #58922, #9177, #100755, #11090, #1283, #128980, #39316, #29466, #41236, #69371, #109303, #19649, #51691, #62799, #124293, #12390, #54258, #94176, #41874, #32709, #2551, #3862, #91603, #103366, #33351, #11750, #4480, #113169, #22235, #13672, #61519, #43811, #123624, #44431, #121696, #53616, #42525, #101427, #104004, #82450, #34639, #84360, #73894, #112546, #74540, #111894, #102072, #14312, #22879, #64075, #83725, #92911, #33976, #113828, #1921, #24156, #62162, #23497, #102698, #81769, #114456, #73251, #32059, #71979, #52324, #3231, #92234, #93537, #122365, #72615, #63432, #13011, #52971, #43170, #83086, #123000, #36570, #7065, #116382, #17536, #64711, #104633, #97397, #94824, #5146, #37835, #6406, #7713, #45095, #86270, #37206, #35278, #26097, #77742, #84992, #56173, #54888, #45734, #77121, #47029, #96106, #86927, #126870, #14936, #117015, #25419, #76482, #66004, #57486, #127513, #47668, #85644, #5773, #15604, #46356, #26730, #126218, #124930, #87569, #75184, #125560, #115083, #35905, #65346, #95469, #27349, #66640, #105292, #67255, #106565, #107214, #24799, #16867, #55552, #75815, #56806, #105934, #115742, #16237, #96738, #67935, #80351, #89514, #48961, #119611, #29962, #60710, #69880, #8363, #88871, #107862, #98676, #28021, #58772, #120276, #19476, #88195, #10312, #18186, #99990, #58134, #49611, #468, #128156, #118974, #41087, #98043, #59438, #20134, #29315, #50884, #30616, #128830, #9666, #38506, #9006, #68578, #79690, #108504, #50247, #90803, #100610, #78434, #99347, #1133, #109806, #60076, #129473, #18834, #39794, #90138, #40438, #48304, #10925, #118327, #39156, #28672, #79067, #69216, #109137, #70512, #110437, #20781, #117654, #31256, #63276, #21416, #12862, #62649, #81621, #14158, #32558, #113018, #54104, #120903, #122208, #94024, #33815, #72462, #31892, #23336, #71816, #52811, #101268, #112387, #71160, #103200, #113669, #111734, #102548, #92081, #61352, #22084, #22730, #11598, #62003, #101918, #103853, #24002, #43656, #92746, #4326, #111062, #63928, #3077, #51540, #91445, #121540, #43028, #80988, #83578, #82931, #122844, #33196, #12231, #73102, #1765, #41726, #52174, #2399, #42359, #73729, #82284, #13519, #53471, #93387, #3706, #123474, #96583, #35754, #106420, #115581, #26582, #14784, #5626, #54731, #75660, #56655, #6905, #35128, #76325, #17377, #84196, #85495, #57328, #126717, #25939, #124778, #124123, #34480, #46210, #116234, #126054, #65844, #74387, #125420, #75034, #105784, #55394, #114308, #114940, #16085, #104486, #25264, #65186, #67106, #76967, #46871, #107054, #66489, #6267, #16724, #44272, #24645, #105126, #45581, #97245, #15446, #56021, #95958, #86115, #86772, #36414, #64559, #37052, #94661, #116871, #4983, #27212, #95320, #44935, #84846, #69071, #27865, #39010, #47515, #39650, #40272, #78920, #118173, #28518, #88718, #110290, #99842, #118822, #29172, #108980, #68427, #80198, #10161, #19318, #60571, #37694, #108350, #78275, #79549, #77592, #49463, #59284, #87415, #127365, #8214, #50106, #98515, #8851, #89994, #29802, #99193, #18685, #9516, #30465, #117497, #57979, #120118, #58629, #311, #20633, #70367, #48810, #128678, #127998, #89370, #129316, #119451, #67783, #7564, #107715, #69726, #109654, #48156, #19985, #59930, #18033, #97886, #88041, #38345, #63119, #72313, #31733, #102412, #12715, #43502, #52650, #112231, #82784, #62499, #93237, #10767, #41574, #103039, #2252, #71020, #122688, #50725, #33043, #40935, #32409, #112875, #110919, #101766, #23856, #80843, #42203, #980, #121395, #73570, #3559, #71654, #22581, #12084, #53318, #23190, #91943, #72948, #82120, #13372, #21256, #61850, #61195, #122056, #83421, #123335, #91294, #120756, #33669, #92587, #113507, #100469, #90649, #111581, #2926, #101117, #21925, #51394, #42872, #1614, #31108, #11442, #81482, #52026, #95165, #36896, #14005, #46069, #4182, #125266, #76173, #74235, #84693, #104337, #25772, #44127, #95803, #65032, #126562, #115409, #35607, #86623, #45428, #64407, #76816, #15287, #6120, #116722, #103703, #104956, #63779, #16576, #75508, #85964, #65696, #56516, #53953, #93875, #6741, #84037, #123966, #34331, #96431, #124624, #44787, #54574, #5472, #105633, #15934, #114162, #46708, #24490, #14644, #25126, #94503, #85339, #116086, #26429, #4827, #34978, #66337, #55872, #106269, #125891, #36255, #74882, #114789, #55246, #67616, #118659, #7407, #59111, #49309, #162, #99684, #37542, #58478, #40114, #99030, #80031, #66967, #68266, #27069, #109494, #18529, #107563, #9360, #17880, #88554, #47356, #98366, #106901, #17205, #108191, #57820, #48641, #38176, #97096, #97732, #8687, #87260, #8059, #48006, #49953, #59776, #119301, #128521, #57165, #127213, #10003, #77452, #39494, #87895, #28363, #127841, #89204, #78106, #38852, #117339, #78764, #27693, #129162, #89843, #29013, #118015, #68915, #108832, #19152, #29644, #79399, #69556, #19833, #13206, #23048, #82625, #11926, #43345, #20476, #62967, #60416, #2749, #10618, #112723, #42049, #31581, #72797, #42715, #111405, #52496, #61699, #102258, #93089, #81956, #121246, #119960, #53158, #2099, #70217, #122541, #91785, #51240, #121886, #32246, #102878, #72158, #112075, #12564, #22423, #3402, #30312, #110136, #100323, #21766, #90477, #92425, #50561, #32886, #823, #51871, #40780, #80689, #71493, #120601, #30950, #101616, #70860, #11283, #110768, #21104, #61031, #62338, #100948, #91142, #1460, #41417, #81329, #4035, #104180, #34161, #45270, #74077, #105474, #56359, #26274, #93719, #114634, #96274, #35453, #25604, #24975, #6583, #43986, #85182, #125111, #66179, #75352, #95014, #65539, #115254, #76003, #123189, #33524, #106113, #45916, #64885, #104803, #15128, #14489, #55082, #16411, #73422, #83885, #113351 ), #15788, .F. ) ;
#45081=FACE_OUTER_BOUND ( 'NONE', #100463, .T. ) ;
#45082=CIRCLE ( 'NONE', #11612, 0.06509327318403745899 ) ;
#45083=FACE_OUTER_BOUND ( 'NONE', #22396, .T. ) ;
#45084=CARTESIAN_POINT ( 'NONE',  ( 4.349999999999940137, 2.500000000000000000, -2.611473670974877592 ) ) ;
#45085=VERTEX_POINT ( 'NONE', #5325 ) ;
#45086=AXIS2_PLACEMENT_3D ( 'NONE', #55882, #34987, #114801 ) ;
#45087=CIRCLE ( 'NONE', #26202, 0.06509327318403745899 ) ;
#45088=DIRECTION ( 'NONE',  ( -4.274815082592931898E-19, -0.9999939076577903929, -0.003490651415223739937 ) ) ;
#45089=ORIENTED_EDGE ( 'NONE', *, *, #124799, .F. ) ;
#45090=ORIENTED_EDGE ( 'NONE', *, *, #811, .T. ) ;
#45091=ORIENTED_EDGE ( 'NONE', *, *, #37766, .F. ) ;
#45092=VERTEX_POINT ( 'NONE', #63623 ) ;
#45093=EDGE_CURVE ( 'NONE', #74899, #104652, #83266, .T. ) ;
#45094=CARTESIAN_POINT ( 'NONE',  ( -1.050000000000038236, 2.500000000000000000, -1.818653347947326138 ) ) ;
#45095=FACE_BOUND ( 'NONE', #86085, .T. ) ;
#45096=DIRECTION ( 'NONE',  ( -0.000000000000000000, 1.000000000000000000, -0.000000000000000000 ) ) ;
#45097=AXIS2_PLACEMENT_3D ( 'NONE', #24139, #12372, #81751 ) ;
#45098=CIRCLE ( 'NONE', #124520, 0.06509327318403745899 ) ;
#45099=ORIENTED_EDGE ( 'NONE', *, *, #38941, .F. ) ;
#45100=CARTESIAN_POINT ( 'NONE',  ( 21.24754738303277435, 0.7337760880902300942, 4.182111650399361835 ) ) ;
#45101=PLANE ( 'NONE',  #68715 ) ;
#45102=EDGE_LOOP ( 'NONE', ( #105239, #61897 ) ) ;
#45103=DIRECTION ( 'NONE',  ( 0.000000000000000000, 0.000000000000000000, 1.000000000000000000 ) ) ;
#45104=CARTESIAN_POINT ( 'NONE',  ( -7.500000000000016875, 2.500000000000000000, -3.737306695894649700 ) ) ;
#45105=AXIS2_PLACEMENT_3D ( 'NONE', #95788, #46055, #106253 ) ;
#45106=AXIS2_PLACEMENT_3D ( 'NONE', #85190, #103557, #4045 ) ;
#45107=EDGE_LOOP ( 'NONE', ( #2739, #116063 ) ) ;
#45108=PLANE ( 'NONE',  #100881 ) ;
#45109=LINE ( 'NONE', #76499, #70501 ) ;
#45110=ORIENTED_EDGE ( 'NONE', *, *, #67084, .T. ) ;
#45111=EDGE_CURVE ( 'NONE', #117010, #94365, #39132, .T. ) ;
#45112=CARTESIAN_POINT ( 'NONE',  ( -12.09999999999999432, 12.50000000000000000, 3.637306695894644726 ) ) ;
#45114=DIRECTION ( 'NONE',  ( 0.000000000000000000, 1.000000000000000000, 0.000000000000000000 ) ) ;
#45115=VERTEX_POINT ( 'NONE', #114011 ) ;
#45116=ORIENTED_EDGE ( 'NONE', *, *, #85385, .F. ) ;
#45117=DIRECTION ( 'NONE',  ( -0.000000000000000000, -1.000000000000000000, -0.000000000000000000 ) ) ;
#45118=EDGE_CURVE ( 'NONE', #13831, #97216, #24336, .T. ) ;
#45119=ORIENTED_EDGE ( 'NONE', *, *, #117058, .T. ) ;
#45120=DIRECTION ( 'NONE',  ( -0.000000000000000000, -1.000000000000000000, -0.000000000000000000 ) ) ;
#45121=DIRECTION ( 'NONE',  ( 0.000000000000000000, -0.000000000000000000, 1.000000000000000000 ) ) ;
#45122=CIRCLE ( 'NONE', #55579, 0.06509327318403745899 ) ;
#45123=VERTEX_POINT ( 'NONE', #64249 ) ;
#45124=CIRCLE ( 'NONE', #120340, 0.06509327318403745899 ) ;
#45125=DIRECTION ( 'NONE',  ( -0.000000000000000000, -1.000000000000000000, -0.000000000000000000 ) ) ;
#45126=LINE ( 'NONE', #53011, #127766 ) ;
#45127=CARTESIAN_POINT ( 'NONE',  ( -3.750000000000029310, 2.500000000000000000, -7.288010851410854585 ) ) ;
#45128=EDGE_CURVE ( 'NONE', #7788, #99762, #13956, .T. ) ;
#45129=ADVANCED_FACE ( 'NONE', ( #115930 ), #32859, .T. ) ;
#45130=DIRECTION ( 'NONE',  ( 0.000000000000000000, 0.000000000000000000, -1.000000000000000000 ) ) ;
#45131=ADVANCED_FACE ( 'NONE', ( #36091 ), #34822, .T. ) ;
#45132=EDGE_CURVE ( 'NONE', #114231, #90411, #60728, .T. ) ;
#45133=EDGE_CURVE ( 'NONE', #114688, #101225, #80879, .T. ) ;
#45134=DIRECTION ( 'NONE',  ( -0.000000000000000000, -1.000000000000000000, -0.000000000000000000 ) ) ;
#45135=VERTEX_POINT ( 'NONE', #58320 ) ;
#45136=EDGE_LOOP ( 'NONE', ( #66402, #40754 ) ) ;
#45137=CARTESIAN_POINT ( 'NONE',  ( -1.250000000000001110, 12.50000000000000000, -2.165063509461101710 ) ) ;
#45138=CARTESIAN_POINT ( 'NONE',  ( 2.299999999999946976, 12.50000000000000000, 4.676537180435972552 ) ) ;
#45139=CARTESIAN_POINT ( 'NONE',  ( -1.900000000000035438, 12.50000000000000000, 4.048810130592458201 ) ) ;
#45140=AXIS2_PLACEMENT_3D ( 'NONE', #99134, #70957, #69011 ) ;
#45141=EDGE_LOOP ( 'NONE', ( #22797, #108149 ) ) ;
#45142=EDGE_LOOP ( 'NONE', ( #86486, #9528, #81615, #12953 ) ) ;
#45143=ORIENTED_EDGE ( 'NONE', *, *, #67973, .T. ) ;
#45144=EDGE_CURVE ( 'NONE', #57084, #2830, #93391, .T. ) ;
#45145=DIRECTION ( 'NONE',  ( 0.000000000000000000, 0.000000000000000000, 1.000000000000000000 ) ) ;
#45146=ADVANCED_FACE ( 'NONE', ( #18368 ), #66378, .T. ) ;
#45147=AXIS2_PLACEMENT_3D ( 'NONE', #128592, #58549, #27771 ) ;
#45148=DIRECTION ( 'NONE',  ( -0.000000000000000000, 1.000000000000000000, -0.000000000000000000 ) ) ;
#45149=CIRCLE ( 'NONE', #22175, 0.1000000000000000472 ) ;
#45150=EDGE_CURVE ( 'NONE', #49498, #9133, #110109, .T. ) ;
#45151=DIRECTION ( 'NONE',  ( 0.000000000000000000, 1.000000000000000000, 0.000000000000000000 ) ) ;
#45153=DIRECTION ( 'NONE',  ( 0.000000000000000000, 1.000000000000000000, 0.000000000000000000 ) ) ;
#45154=DIRECTION ( 'NONE',  ( -0.000000000000000000, 1.000000000000000000, -0.000000000000000000 ) ) ;
#45155=LINE ( 'NONE', #124988, #82011 ) ;
#45156=CIRCLE ( 'NONE', #107829, 0.1000000000000002554 ) ;
#45157=CARTESIAN_POINT ( 'NONE',  ( -3.749999999999991118, 12.50000000000000000, -2.230156782645139391 ) ) ;
#45158=DIRECTION ( 'NONE',  ( 0.000000000000000000, 1.000000000000000000, 0.000000000000000000 ) ) ;
#45159=CARTESIAN_POINT ( 'NONE',  ( -9.800000000000004263, 2.500000000000000000, 3.983716857408420076 ) ) ;
#45160=VERTEX_POINT ( 'NONE', #41105 ) ;
#45161=FACE_OUTER_BOUND ( 'NONE', #128203, .T. ) ;
#45162=ORIENTED_EDGE ( 'NONE', *, *, #100595, .F. ) ;
#45163=VERTEX_POINT ( 'NONE', #118500 ) ;
#45164=CARTESIAN_POINT ( 'NONE',  ( -4.150000000000025224, 12.50000000000000000, 5.802370205355744659 ) ) ;
#45165=FACE_OUTER_BOUND ( 'NONE', #15422, .T. ) ;
#45166=CONICAL_SURFACE ( 'NONE', #34715, 0.1000000000000000472, 0.003490658503988666988 ) ;
#45167=CARTESIAN_POINT ( 'NONE',  ( -13.09999999999999076, 12.50000000000000000, 4.676537180435972552 ) ) ;
#45168=DIRECTION ( 'NONE',  ( 0.000000000000000000, 0.000000000000000000, -1.000000000000000000 ) ) ;
#45169=LINE ( 'NONE', #125006, #48599 ) ;
#45170=FACE_OUTER_BOUND ( 'NONE', #23229, .T. ) ;
#45171=DIRECTION ( 'NONE',  ( 0.000000000000000000, 1.000000000000000000, 0.000000000000000000 ) ) ;
#45172=VERTEX_POINT ( 'NONE', #38688 ) ;
#45173=CARTESIAN_POINT ( 'NONE',  ( -2.900000000000029221, 2.500000000000000000, -4.230127018922201998 ) ) ;
#45174=VECTOR ( 'NONE', #15627, 1000.000000000000000 ) ;
#45175=CIRCLE ( 'NONE', #124587, 0.09999999999999999167 ) ;
#45176=VECTOR ( 'NONE', #104325, 1000.000000000000000 ) ;
#45177=DIRECTION ( 'NONE',  ( 0.000000000000000000, 0.000000000000000000, -1.000000000000000000 ) ) ;
#45178=ORIENTED_EDGE ( 'NONE', *, *, #48109, .T. ) ;
#45179=ORIENTED_EDGE ( 'NONE', *, *, #92304, .F. ) ;
#45180=VECTOR ( 'NONE', #115223, 1000.000000000000000 ) ;
#45181=VERTEX_POINT ( 'NONE', #8532 ) ;
#45182=EDGE_CURVE ( 'NONE', #55240, #127628, #129106, .T. ) ;
#45183=ORIENTED_EDGE ( 'NONE', *, *, #101211, .F. ) ;
#45184=DIRECTION ( 'NONE',  ( -0.000000000000000000, 1.000000000000000000, -0.000000000000000000 ) ) ;
#45185=DIRECTION ( 'NONE',  ( 0.000000000000000000, -0.9999939076577903929, 0.003490651415223739937 ) ) ;
#45186=CONICAL_SURFACE ( 'NONE', #80790, 0.1000000000000002554, 0.003490658503988666988 ) ;
#45187=EDGE_CURVE ( 'NONE', #6862, #48547, #49682, .T. ) ;
#45188=CARTESIAN_POINT ( 'NONE',  ( 16.55874544816221317, -0.4845305829210151960, -6.091953208799018249 ) ) ;
#45189=DIRECTION ( 'NONE',  ( 0.000000000000000000, -0.9999939076577903929, 0.003490651415223739937 ) ) ;
#45190=AXIS2_PLACEMENT_3D ( 'NONE', #109352, #40, #40647 ) ;
#45191=CIRCLE ( 'NONE', #76488, 0.06509327318403745899 ) ;
#45192=EDGE_CURVE ( 'NONE', #96334, #68282, #57983, .T. ) ;
#45193=DIRECTION ( 'NONE',  ( 0.000000000000000000, 0.000000000000000000, 1.000000000000000000 ) ) ;
#45194=ORIENTED_EDGE ( 'NONE', *, *, #74399, .F. ) ;
#45195=FACE_OUTER_BOUND ( 'NONE', #106717, .T. ) ;
#45196=DIRECTION ( 'NONE',  ( 0.000000000000000000, -0.9999939076577903929, 0.003490651415223739937 ) ) ;
#45197=EDGE_CURVE ( 'NONE', #126533, #92856, #126939, .T. ) ;
#45198=CARTESIAN_POINT ( 'NONE',  ( -10.65000000000000213, 12.50000000000000000, 6.841600689897072485 ) ) ;
#45199=ORIENTED_EDGE ( 'NONE', *, *, #57727, .F. ) ;
#45201=ORIENTED_EDGE ( 'NONE', *, *, #12627, .F. ) ;
#45203=CARTESIAN_POINT ( 'NONE',  ( -10.80000000000000249, 12.50000000000000000, -4.330127018922197202 ) ) ;
#45204=CARTESIAN_POINT ( 'NONE',  ( -9.150000000000009237, 2.500000000000000000, -2.857883832488653741 ) ) ;
#45205=VERTEX_POINT ( 'NONE', #47852 ) ;
#45206=CARTESIAN_POINT ( 'NONE',  ( 4.349999999999941025, 2.500000000000000000, -6.148780366869526226 ) ) ;
#45207=DIRECTION ( 'NONE',  ( 0.000000000000000000, 0.000000000000000000, -1.000000000000000000 ) ) ;
#45208=CARTESIAN_POINT ( 'NONE',  ( -2.300000000000033573, 2.500000000000000000, 0.3464101615137735735 ) ) ;
#45209=DIRECTION ( 'NONE',  ( 0.000000000000000000, 0.000000000000000000, -1.000000000000000000 ) ) ;
#45210=EDGE_CURVE ( 'NONE', #40173, #16061, #9945, .T. ) ;
#45211=DIRECTION ( 'NONE',  ( 0.000000000000000000, -0.9999939076577903929, 0.003490651415223739937 ) ) ;
#45212=EDGE_LOOP ( 'NONE', ( #94853, #23370, #103466, #74771 ) ) ;
#45214=DIRECTION ( 'NONE',  ( -0.000000000000000000, 1.000000000000000000, -0.000000000000000000 ) ) ;
#45215=CONICAL_SURFACE ( 'NONE', #22239, 0.1000000000000000472, 0.003490658503988666988 ) ;
#45216=ORIENTED_EDGE ( 'NONE', *, *, #42393, .F. ) ;
#45217=ORIENTED_EDGE ( 'NONE', *, *, #35112, .F. ) ;
#45218=ORIENTED_EDGE ( 'NONE', *, *, #69944, .T. ) ;
#45220=FACE_BOUND ( 'NONE', #50224, .T. ) ;
#45221=CARTESIAN_POINT ( 'NONE',  ( -9.600000000000008527, 12.50000000000000000, -4.957854068765712441 ) ) ;
#45222=CARTESIAN_POINT ( 'NONE',  ( -1.050000000000038236, 12.50000000000000000, -6.083687093685488989 ) ) ;
#45223=AXIS2_PLACEMENT_3D ( 'NONE', #7503, #69003, #27152 ) ;
#45225=ADVANCED_FACE ( 'NONE', ( #77294 ), #17044, .T. ) ;
#45226=EDGE_LOOP ( 'NONE', ( #39837, #57569, #90228, #59681 ) ) ;
#45227=DIRECTION ( 'NONE',  ( 0.000000000000000000, 1.000000000000000000, 0.000000000000000000 ) ) ;
#45228=DIRECTION ( 'NONE',  ( -4.274815082592931898E-19, -0.9999939076577903929, -0.003490651415223739937 ) ) ;
#45229=PLANE ( 'NONE',  #67485 ) ;
#45230=CARTESIAN_POINT ( 'NONE',  ( -11.64999999999999680, 2.500000000000000000, 7.088010851410848190 ) ) ;
#45231=EDGE_LOOP ( 'NONE', ( #109707, #94444 ) ) ;
#45232=AXIS2_PLACEMENT_3D ( 'NONE', #98289, #38098, #77378 ) ;
#45233=CIRCLE ( 'NONE', #97537, 0.06509327318403745899 ) ;
#45234=DIRECTION ( 'NONE',  ( -4.274815082592931898E-19, -0.9999939076577903929, -0.003490651415223739937 ) ) ;
#45236=ORIENTED_EDGE ( 'NONE', *, *, #76632, .T. ) ;
#45237=DIRECTION ( 'NONE',  ( -0.000000000000000000, -1.000000000000000000, -0.000000000000000000 ) ) ;
#45238=EDGE_CURVE ( 'NONE', #108508, #106998, #7791, .T. ) ;
#45239=VERTEX_POINT ( 'NONE', #97574 ) ;
#45240=FACE_BOUND ( 'NONE', #127236, .T. ) ;
#45241=DIRECTION ( 'NONE',  ( 0.000000000000000000, 0.000000000000000000, 1.000000000000000000 ) ) ;
#45242=EDGE_LOOP ( 'NONE', ( #63834, #102153 ) ) ;
#45243=DIRECTION ( 'NONE',  ( -4.274815082592931898E-19, -0.9999939076577903929, -0.003490651415223739937 ) ) ;
#45244=FACE_OUTER_BOUND ( 'NONE', #58978, .T. ) ;
#45245=ORIENTED_EDGE ( 'NONE', *, *, #77643, .T. ) ;
#45246=ORIENTED_EDGE ( 'NONE', *, *, #75293, .F. ) ;
#45249=LINE ( 'NONE', #119141, #59461 ) ;
#45250=FACE_OUTER_BOUND ( 'NONE', #58284, .T. ) ;
#45251=CONICAL_SURFACE ( 'NONE', #76644, 0.1000000000000002554, 0.003490658503988666988 ) ;
#45252=CIRCLE ( 'NONE', #61984, 0.06509327318403745899 ) ;
#45253=EDGE_CURVE ( 'NONE', #80196, #90044, #74696, .T. ) ;
#45254=DIRECTION ( 'NONE',  ( 0.000000000000000000, 0.000000000000000000, -1.000000000000000000 ) ) ;
#45255=DIRECTION ( 'NONE',  ( 0.000000000000000000, 0.000000000000000000, 1.000000000000000000 ) ) ;
#45256=DIRECTION ( 'NONE',  ( 0.000000000000000000, 1.000000000000000000, 0.000000000000000000 ) ) ;
#45257=CIRCLE ( 'NONE', #70301, 0.06509327318403745899 ) ;
#45258=CARTESIAN_POINT ( 'NONE',  ( -7.050000000000013145, 2.500000000000000000, 2.065063509461097624 ) ) ;
#45259=CIRCLE ( 'NONE', #116341, 0.1000000000000002554 ) ;
#45260=EDGE_LOOP ( 'NONE', ( #34885, #93551 ) ) ;
#45261=AXIS2_PLACEMENT_3D ( 'NONE', #42526, #33353, #93538 ) ;
#45262=EDGE_CURVE ( 'NONE', #126164, #71809, #87746, .T. ) ;
#45263=VERTEX_POINT ( 'NONE', #66813 ) ;
#45264=LINE ( 'NONE', #54420, #121777 ) ;
#45265=CARTESIAN_POINT ( 'NONE',  ( -7.700000000000016165, 2.500000000000000000, 0.2464101615137735679 ) ) ;
#45266=DIRECTION ( 'NONE',  ( 0.000000000000000000, -0.000000000000000000, 1.000000000000000000 ) ) ;
#45267=CARTESIAN_POINT ( 'NONE',  ( 1.899999999999949507, 12.50000000000000000, 4.741630453620009789 ) ) ;
#45268=VERTEX_POINT ( 'NONE', #7900 ) ;
#45269=EDGE_LOOP ( 'NONE', ( #1633, #88865, #97057, #125155 ) ) ;
#45270=FACE_BOUND ( 'NONE', #125954, .T. ) ;
#45271=ORIENTED_EDGE ( 'NONE', *, *, #128067, .F. ) ;
#45272=FACE_OUTER_BOUND ( 'NONE', #76078, .T. ) ;
#45273=DIRECTION ( 'NONE',  ( 0.000000000000000000, 0.000000000000000000, 1.000000000000000000 ) ) ;
#45274=AXIS2_PLACEMENT_3D ( 'NONE', #116055, #26405, #68238 ) ;
#45275=VERTEX_POINT ( 'NONE', #106744 ) ;
#45276=CARTESIAN_POINT ( 'NONE',  ( -11.44999999999999751, 2.500000000000000000, -6.741600689897073728 ) ) ;
#45277=EDGE_CURVE ( 'NONE', #9179, #15257, #14039, .T. ) ;
#45278=DIRECTION ( 'NONE',  ( 0.000000000000000000, 1.000000000000000000, 0.000000000000000000 ) ) ;
#45279=CARTESIAN_POINT ( 'NONE',  ( -9.200000000000006395, 2.500000000000000000, 4.330127018922196314 ) ) ;
#45280=AXIS2_PLACEMENT_3D ( 'NONE', #96625, #74440, #75079 ) ;
#45281=VECTOR ( 'NONE', #57003, 1000.000000000000000 ) ;
#45282=CARTESIAN_POINT ( 'NONE',  ( -4.400000000000025224, 2.500000000000000000, 4.083716857408420609 ) ) ;
#45283=DIRECTION ( 'NONE',  ( 0.000000000000000000, 0.000000000000000000, 1.000000000000000000 ) ) ;
#45284=CARTESIAN_POINT ( 'NONE',  ( -7.300000000000018474, 2.500000000000000000, 0.3464101615137735735 ) ) ;
#45285=ADVANCED_FACE ( 'NONE', ( #50914 ), #16185, .T. ) ;
#45286=ADVANCED_FACE ( 'NONE', ( #4345 ), #26585, .T. ) ;
#45288=LINE ( 'NONE', #87124, #33901 ) ;
#45289=EDGE_CURVE ( 'NONE', #83265, #14140, #62020, .T. ) ;
#45290=EDGE_CURVE ( 'NONE', #117196, #49455, #91464, .T. ) ;
#45291=DIRECTION ( 'NONE',  ( -0.000000000000000000, 1.000000000000000000, -0.000000000000000000 ) ) ;
#45292=ORIENTED_EDGE ( 'NONE', *, *, #37917, .T. ) ;
#45293=VERTEX_POINT ( 'NONE', #63947 ) ;
#45294=CARTESIAN_POINT ( 'NONE',  ( 3.099999999999945466, 2.500000000000000000, -4.083716857408426826 ) ) ;
#45295=VERTEX_POINT ( 'NONE', #31911 ) ;
#45296=EDGE_CURVE ( 'NONE', #7787, #85940, #101939, .T. ) ;
#45297=CARTESIAN_POINT ( 'NONE',  ( -2.500000000000030642, 2.500000000000000000, -5.022947341949754119 ) ) ;
#45298=EDGE_CURVE ( 'NONE', #29719, #107907, #3100, .T. ) ;
#45299=ORIENTED_EDGE ( 'NONE', *, *, #47779, .T. ) ;
#45300=EDGE_LOOP ( 'NONE', ( #67102, #77734, #128558, #35335 ) ) ;
#45301=EDGE_LOOP ( 'NONE', ( #106001, #66241, #78393, #74263 ) ) ;
#45302=EDGE_CURVE ( 'NONE', #111299, #116195, #45474, .T. ) ;
#45303=LINE ( 'NONE', #7279, #102298 ) ;
#45304=EDGE_CURVE ( 'NONE', #71756, #117403, #41267, .T. ) ;
#45305=EDGE_CURVE ( 'NONE', #23899, #98477, #32959, .T. ) ;
#45306=DIRECTION ( 'NONE',  ( -0.000000000000000000, 1.000000000000000000, -0.000000000000000000 ) ) ;
#45307=PLANE ( 'NONE',  #74377 ) ;
#45309=LINE ( 'NONE', #76047, #43368 ) ;
#45310=VERTEX_POINT ( 'NONE', #81642 ) ;
#45311=ADVANCED_FACE ( 'NONE', ( #33216 ), #120676, .T. ) ;
#45312=LINE ( 'NONE', #115292, #118731 ) ;
#45313=EDGE_LOOP ( 'NONE', ( #27610, #42648, #128827, #4034 ) ) ;
#45314=AXIS2_PLACEMENT_3D ( 'NONE', #30162, #70075, #59638 ) ;
#45315=ORIENTED_EDGE ( 'NONE', *, *, #121508, .T. ) ;
#45316=EDGE_LOOP ( 'NONE', ( #100224, #128356 ) ) ;
#45317=AXIS2_PLACEMENT_3D ( 'NONE', #18927, #9123, #49069 ) ;
#45318=LINE ( 'NONE', #23739, #56854 ) ;
#45319=ORIENTED_EDGE ( 'NONE', *, *, #84897, .F. ) ;
#45320=EDGE_LOOP ( 'NONE', ( #120747, #36185, #81592, #31266 ) ) ;
#45321=EDGE_LOOP ( 'NONE', ( #42238, #3979 ) ) ;
#45323=AXIS2_PLACEMENT_3D ( 'NONE', #51168, #89785, #119244 ) ;
#45324=CONICAL_SURFACE ( 'NONE', #13902, 0.09999999999999982514, 0.003490658503988666988 ) ;
#45325=DIRECTION ( 'NONE',  ( 0.000000000000000000, 0.000000000000000000, 1.000000000000000000 ) ) ;
#45326=DIRECTION ( 'NONE',  ( 0.000000000000000000, 0.000000000000000000, 1.000000000000000000 ) ) ;
#45327=DIRECTION ( 'NONE',  ( 0.000000000000000000, 0.000000000000000000, 1.000000000000000000 ) ) ;
#45328=CARTESIAN_POINT ( 'NONE',  ( 5.399999999999932854, 2.500000000000000000, 5.122947341949749323 ) ) ;
#45329=DIRECTION ( 'NONE',  ( 0.000000000000000000, 0.000000000000000000, 1.000000000000000000 ) ) ;
#45330=ORIENTED_EDGE ( 'NONE', *, *, #122387, .T. ) ;
#45331=VECTOR ( 'NONE', #35465, 1000.000000000000000 ) ;
#45332=CARTESIAN_POINT ( 'NONE',  ( 9.549999999999915445, 12.50000000000000000, -2.165063509461101710 ) ) ;
#45333=AXIS2_PLACEMENT_3D ( 'NONE', #69472, #109403, #11195 ) ;
#45334=CONICAL_SURFACE ( 'NONE', #97638, 0.1000000000000000472, 0.003490658503988666988 ) ;
#45335=ORIENTED_EDGE ( 'NONE', *, *, #12200, .F. ) ;
#45336=DIRECTION ( 'NONE',  ( 0.000000000000000000, 1.000000000000000000, 0.000000000000000000 ) ) ;
#45337=CIRCLE ( 'NONE', #118468, 0.06509327318403745899 ) ;
#45338=ORIENTED_EDGE ( 'NONE', *, *, #111132, .T. ) ;
#45340=ORIENTED_EDGE ( 'NONE', *, *, #121149, .T. ) ;
#45341=ORIENTED_EDGE ( 'NONE', *, *, #77573, .F. ) ;
#45342=DIRECTION ( 'NONE',  ( 0.000000000000000000, 0.000000000000000000, 1.000000000000000000 ) ) ;
#45343=DIRECTION ( 'NONE',  ( 0.000000000000000000, -0.9999939076577903929, 0.003490651415223739937 ) ) ;
#45344=EDGE_CURVE ( 'NONE', #112557, #97087, #114399, .T. ) ;
#45345=DIRECTION ( 'NONE',  ( 0.000000000000000000, 1.000000000000000000, 0.000000000000000000 ) ) ;
#45346=ADVANCED_FACE ( 'NONE', ( #74410 ), #85152, .T. ) ;
#45347=CARTESIAN_POINT ( 'NONE',  ( -12.89999999999999147, 2.500000000000000000, 5.022947341949748790 ) ) ;
#45348=ORIENTED_EDGE ( 'NONE', *, *, #20031, .T. ) ;
#45349=CARTESIAN_POINT ( 'NONE',  ( -1.700000000000035261, 2.500000000000000000, 4.330127018922196314 ) ) ;
#45350=FACE_OUTER_BOUND ( 'NONE', #106754, .T. ) ;
#45351=DIRECTION ( 'NONE',  ( 0.000000000000000000, 0.000000000000000000, -1.000000000000000000 ) ) ;
#45352=AXIS2_PLACEMENT_3D ( 'NONE', #73126, #82312, #122237 ) ;
#45353=DIRECTION ( 'NONE',  ( -0.000000000000000000, 1.000000000000000000, -0.000000000000000000 ) ) ;
#45354=CONICAL_SURFACE ( 'NONE', #18433, 0.1000000000000002554, 0.003490658503988666988 ) ;
#45355=ADVANCED_FACE ( 'NONE', ( #84214 ), #28742, .T. ) ;
#45356=DIRECTION ( 'NONE',  ( 0.000000000000000000, 0.000000000000000000, 1.000000000000000000 ) ) ;
#45357=ORIENTED_EDGE ( 'NONE', *, *, #58471, .T. ) ;
#45358=EDGE_CURVE ( 'NONE', #99447, #104181, #64226, .T. ) ;
#45359=CIRCLE ( 'NONE', #110192, 0.09999999999999982514 ) ;
#45360=EDGE_LOOP ( 'NONE', ( #14549, #21692 ) ) ;
#45361=CIRCLE ( 'NONE', #1419, 0.06509327318403745899 ) ;
#45362=EDGE_LOOP ( 'NONE', ( #39311, #95013 ) ) ;
#45363=CONICAL_SURFACE ( 'NONE', #89263, 0.1000000000000002554, 0.003490658503988666988 ) ;
#45364=DIRECTION ( 'NONE',  ( 0.000000000000000000, -0.9999939076577903929, 0.003490651415223739937 ) ) ;
#45365=DIRECTION ( 'NONE',  ( -0.000000000000000000, 1.000000000000000000, -0.000000000000000000 ) ) ;
#45366=AXIS2_PLACEMENT_3D ( 'NONE', #127150, #19086, #6681 ) ;
#45368=CARTESIAN_POINT ( 'NONE',  ( 8.749999999999920064, 2.500000000000000000, 5.702370205355745014 ) ) ;
#45369=AXIS2_PLACEMENT_3D ( 'NONE', #13715, #1324, #22284 ) ;
#45370=CARTESIAN_POINT ( 'NONE',  ( 4.349999999999941025, 12.50000000000000000, -6.148780366869526226 ) ) ;
#45371=CARTESIAN_POINT ( 'NONE',  ( 9.999999999999911182, 12.50000000000000000, -3.637306695894650055 ) ) ;
#45372=CARTESIAN_POINT ( 'NONE',  ( 0.4499999999999569344, 2.500000000000000000, -2.265063509461101798 ) ) ;
#45373=EDGE_LOOP ( 'NONE', ( #103381, #54213 ) ) ;
#45374=AXIS2_PLACEMENT_3D ( 'NONE', #110739, #30917, #81922 ) ;
#45375=AXIS2_PLACEMENT_3D ( 'NONE', #30514, #70414, #91984 ) ;
#45376=AXIS2_PLACEMENT_3D ( 'NONE', #14343, #14970, #54286 ) ;
#45377=DIRECTION ( 'NONE',  ( 0.000000000000000000, 0.000000000000000000, -1.000000000000000000 ) ) ;
#45378=CARTESIAN_POINT ( 'NONE',  ( 3.349999999999943689, 12.50000000000000000, 1.407149913249508000 ) ) ;
#45379=EDGE_LOOP ( 'NONE', ( #48731, #41530, #3680, #90186 ) ) ;
#45380=DIRECTION ( 'NONE',  ( 0.000000000000000000, 1.000000000000000000, 0.000000000000000000 ) ) ;
#45381=DIRECTION ( 'NONE',  ( -0.000000000000000000, -1.000000000000000000, -0.000000000000000000 ) ) ;
#45382=DIRECTION ( 'NONE',  ( 0.000000000000000000, 0.000000000000000000, 1.000000000000000000 ) ) ;
#45383=EDGE_CURVE ( 'NONE', #37632, #117649, #92102, .T. ) ;
#45384=ORIENTED_EDGE ( 'NONE', *, *, #47244, .F. ) ;
#45385=CARTESIAN_POINT ( 'NONE',  ( 0.7999999999999553024, 12.50000000000000000, -4.330127018922201643 ) ) ;
#45386=EDGE_LOOP ( 'NONE', ( #16739, #25568, #61996, #76980 ) ) ;
#45387=CARTESIAN_POINT ( 'NONE',  ( 0.3999999999999628852, 12.50000000000000000, 0.6928203230275518099 ) ) ;
#45388=DIRECTION ( 'NONE',  ( 0.000000000000000000, 0.000000000000000000, 1.000000000000000000 ) ) ;
#45389=AXIS2_PLACEMENT_3D ( 'NONE', #114966, #102574, #12891 ) ;
#45390=DIRECTION ( 'NONE',  ( 0.000000000000000000, 0.000000000000000000, 1.000000000000000000 ) ) ;
#45391=ORIENTED_EDGE ( 'NONE', *, *, #5232, .F. ) ;
#45393=CARTESIAN_POINT ( 'NONE',  ( -7.500000000000001776, -1.500000000000000000, -8.999999999999998224 ) ) ;
#45394=EDGE_CURVE ( 'NONE', #62921, #64709, #3594, .T. ) ;
#45395=EDGE_CURVE ( 'NONE', #73490, #72875, #54124, .T. ) ;
#45396=EDGE_LOOP ( 'NONE', ( #89023, #103520 ) ) ;
#45397=DIRECTION ( 'NONE',  ( 0.000000000000000000, 0.000000000000000000, 1.000000000000000000 ) ) ;
#45398=CIRCLE ( 'NONE', #32892, 0.06509327318403745899 ) ;
#45399=ORIENTED_EDGE ( 'NONE', *, *, #8203, .T. ) ;
#45400=CIRCLE ( 'NONE', #126875, 0.06509327318403741736 ) ;
#45401=EDGE_LOOP ( 'NONE', ( #110759, #18667 ) ) ;
#45402=DIRECTION ( 'NONE',  ( -0.000000000000000000, 1.000000000000000000, -0.000000000000000000 ) ) ;
#45403=DIRECTION ( 'NONE',  ( 0.000000000000000000, 1.000000000000000000, 0.000000000000000000 ) ) ;
#45404=EDGE_CURVE ( 'NONE', #116963, #111573, #95627, .T. ) ;
#45405=ORIENTED_EDGE ( 'NONE', *, *, #116811, .T. ) ;
#45406=CARTESIAN_POINT ( 'NONE',  ( -4.150000000000025224, 2.500000000000000000, 2.857883832488649301 ) ) ;
#45407=PLANE ( 'NONE',  #69388 ) ;
#45408=EDGE_LOOP ( 'NONE', ( #45938, #82088 ) ) ;
#45409=AXIS2_PLACEMENT_3D ( 'NONE', #126342, #47781, #125672 ) ;
#45410=CIRCLE ( 'NONE', #126972, 0.06509327318403745899 ) ;
#45411=DIRECTION ( 'NONE',  ( 0.000000000000000000, -0.9999939076577903929, 0.003490651415223739937 ) ) ;
#45412=CARTESIAN_POINT ( 'NONE',  ( 2.499999999999945377, 2.500000000000000000, 4.922947341949748257 ) ) ;
#45413=CARTESIAN_POINT ( 'NONE',  ( -2.300000000000033129, 2.500000000000000000, 3.983716857408420076 ) ) ;
#45414=DIRECTION ( 'NONE',  ( 0.000000000000000000, -0.000000000000000000, 1.000000000000000000 ) ) ;
#45415=DIRECTION ( 'NONE',  ( -0.000000000000000000, 1.000000000000000000, -0.000000000000000000 ) ) ;
#45417=AXIS2_PLACEMENT_3D ( 'NONE', #61936, #122779, #41020 ) ;
#45418=AXIS2_PLACEMENT_3D ( 'NONE', #73245, #123616, #113163 ) ;
#45419=AXIS2_PLACEMENT_3D ( 'NONE', #37538, #109490, #22418 ) ;
#45420=EDGE_LOOP ( 'NONE', ( #55312, #38874 ) ) ;
#45421=VERTEX_POINT ( 'NONE', #42377 ) ;
#45422=EDGE_LOOP ( 'NONE', ( #79997, #77685 ) ) ;
#45423=ORIENTED_EDGE ( 'NONE', *, *, #75701, .T. ) ;
#45424=CARTESIAN_POINT ( 'NONE',  ( 7.299999999999927880, 12.50000000000000000, -4.676537180435977881 ) ) ;
#45425=LINE ( 'NONE', #127209, #34525 ) ;
#45426=DIRECTION ( 'NONE',  ( -0.000000000000000000, 1.000000000000000000, -0.000000000000000000 ) ) ;
#45427=ORIENTED_EDGE ( 'NONE', *, *, #17652, .T. ) ;
#45428=FACE_BOUND ( 'NONE', #9710, .T. ) ;
#45429=CARTESIAN_POINT ( 'NONE',  ( 4.599999999999938360, 2.500000000000000000, -2.276824562219559311E-15 ) ) ;
#45430=DIRECTION ( 'NONE',  ( 0.000000000000000000, -0.000000000000000000, 1.000000000000000000 ) ) ;
#45431=DIRECTION ( 'NONE',  ( -0.000000000000000000, 1.000000000000000000, -0.000000000000000000 ) ) ;
#45432=EDGE_CURVE ( 'NONE', #38961, #58403, #78923, .T. ) ;
#45433=DIRECTION ( 'NONE',  ( -0.000000000000000000, -1.000000000000000000, -0.000000000000000000 ) ) ;
#45434=DIRECTION ( 'NONE',  ( 0.000000000000000000, 0.000000000000000000, -1.000000000000000000 ) ) ;
#45435=CARTESIAN_POINT ( 'NONE',  ( 3.349999999999945466, 2.500000000000000000, -2.757883832488654097 ) ) ;
#45436=CARTESIAN_POINT ( 'NONE',  ( -3.350000000000028955, 2.500000000000000000, 5.802370205355744659 ) ) ;
#45437=CARTESIAN_POINT ( 'NONE',  ( 3.149999999999942624, 12.50000000000000000, 6.213873640053559022 ) ) ;
#45438=EDGE_CURVE ( 'NONE', #100139, #112224, #110211, .T. ) ;
#45439=DIRECTION ( 'NONE',  ( 0.000000000000000000, 0.000000000000000000, -1.000000000000000000 ) ) ;
#45440=EDGE_CURVE ( 'NONE', #19106, #60583, #39229, .T. ) ;
#45441=AXIS2_PLACEMENT_3D ( 'NONE', #8543, #48492, #98873 ) ;
#45442=ADVANCED_FACE ( 'NONE', ( #56675 ), #108238, .T. ) ;
#45443=CONICAL_SURFACE ( 'NONE', #103926, 0.1000000000000002554, 0.003490658503988666988 ) ;
#45444=DIRECTION ( 'NONE',  ( 0.000000000000000000, 0.000000000000000000, 1.000000000000000000 ) ) ;
#45445=VERTEX_POINT ( 'NONE', #67130 ) ;
#45446=AXIS2_PLACEMENT_3D ( 'NONE', #99779, #50057, #8797 ) ;
#45447=ORIENTED_EDGE ( 'NONE', *, *, #33778, .T. ) ;
#45448=EDGE_LOOP ( 'NONE', ( #28563, #26857 ) ) ;
#45449=ORIENTED_EDGE ( 'NONE', *, *, #119415, .F. ) ;
#45450=CARTESIAN_POINT ( 'NONE',  ( -2.300000000000033129, 12.50000000000000000, 4.048810130592458201 ) ) ;
#45451=ADVANCED_FACE ( 'NONE', ( #46231 ), #68525, .T. ) ;
#45453=DIRECTION ( 'NONE',  ( -0.000000000000000000, 1.000000000000000000, -0.000000000000000000 ) ) ;
#45455=EDGE_CURVE ( 'NONE', #102121, #116823, #66460, .T. ) ;
#45456=ORIENTED_EDGE ( 'NONE', *, *, #71743, .T. ) ;
#45457=AXIS2_PLACEMENT_3D ( 'NONE', #101125, #30473, #11450 ) ;
#45458=ORIENTED_EDGE ( 'NONE', *, *, #126112, .F. ) ;
#45459=DIRECTION ( 'NONE',  ( 0.000000000000000000, 1.000000000000000000, 0.000000000000000000 ) ) ;
#45460=AXIS2_PLACEMENT_3D ( 'NONE', #57334, #76974, #124789 ) ;
#45461=CONICAL_SURFACE ( 'NONE', #97920, 0.09999999999999999167, 0.003490658503988666988 ) ;
#45462=CONICAL_SURFACE ( 'NONE', #118593, 0.1000000000000000056, 0.003490658503988666988 ) ;
#45463=EDGE_CURVE ( 'NONE', #89563, #38596, #28831, .T. ) ;
#45464=CARTESIAN_POINT ( 'NONE',  ( 3.709550432165976463, -1.499999999999871880, 10.00000000000000178 ) ) ;
#45465=DIRECTION ( 'NONE',  ( 0.000000000000000000, 0.000000000000000000, -1.000000000000000000 ) ) ;
#45466=LINE ( 'NONE', #112902, #71921 ) ;
#45467=CARTESIAN_POINT ( 'NONE',  ( -11.64999999999999680, 2.500000000000000000, 6.595190528383296780 ) ) ;
#45469=EDGE_CURVE ( 'NONE', #118395, #69772, #43424, .T. ) ;
#45470=ORIENTED_EDGE ( 'NONE', *, *, #120822, .T. ) ;
#45471=EDGE_CURVE ( 'NONE', #73598, #112989, #83207, .T. ) ;
#45472=EDGE_LOOP ( 'NONE', ( #88011, #81400 ) ) ;
#45473=AXIS2_PLACEMENT_3D ( 'NONE', #42249, #12758, #2965 ) ;
#45474=CIRCLE ( 'NONE', #116453, 0.1000000000000002554 ) ;
#45475=ORIENTED_EDGE ( 'NONE', *, *, #31336, .F. ) ;
#45476=CARTESIAN_POINT ( 'NONE',  ( 1.849999999999948130, 12.50000000000000000, 6.148780366869520009 ) ) ;
#45477=EDGE_LOOP ( 'NONE', ( #8032, #59705 ) ) ;
#45478=CARTESIAN_POINT ( 'NONE',  ( 6.049999999999932321, 12.50000000000000000, 1.753560074763284016 ) ) ;
#45479=ORIENTED_EDGE ( 'NONE', *, *, #24025, .F. ) ;
#45480=EDGE_LOOP ( 'NONE', ( #75008, #48026 ) ) ;
#45481=CARTESIAN_POINT ( 'NONE',  ( 13.34999999999990017, 12.50000000000000000, 1.472243186433545459 ) ) ;
#45482=CARTESIAN_POINT ( 'NONE',  ( -10.84999999999999964, 12.50000000000000000, 5.737276932171707422 ) ) ;
#45483=CARTESIAN_POINT ( 'NONE',  ( 12.49999999999993960, 2.500000000000000000, -4.330127018922201643 ) ) ;
#45485=LINE ( 'NONE', #46111, #25219 ) ;
#45486=LINE ( 'NONE', #118067, #28872 ) ;
#45487=AXIS2_PLACEMENT_3D ( 'NONE', #20019, #99867, #58653 ) ;
#45488=ORIENTED_EDGE ( 'NONE', *, *, #54287, .F. ) ;
#45489=CARTESIAN_POINT ( 'NONE',  ( -5.200000000000020606, 2.500000000000000000, -0.3464101615137782364 ) ) ;
#45490=ORIENTED_EDGE ( 'NONE', *, *, #79718, .T. ) ;
#45491=DIRECTION ( 'NONE',  ( 0.000000000000000000, 0.000000000000000000, 1.000000000000000000 ) ) ;
#45492=ORIENTED_EDGE ( 'NONE', *, *, #117204, .F. ) ;
#45493=CARTESIAN_POINT ( 'NONE',  ( 7.299999999999926104, 12.50000000000000000, -3.983716857408426293 ) ) ;
#45494=CARTESIAN_POINT ( 'NONE',  ( -13.29999999999999005, 12.50000000000000000, -4.330127018922198978 ) ) ;
#45495=ORIENTED_EDGE ( 'NONE', *, *, #121628, .F. ) ;
#45496=CARTESIAN_POINT ( 'NONE',  ( -9.200000000000006395, 2.500000000000000000, 4.230127018922196669 ) ) ;
#45497=DIRECTION ( 'NONE',  ( 0.000000000000000000, 1.000000000000000000, 0.000000000000000000 ) ) ;
#45498=ORIENTED_EDGE ( 'NONE', *, *, #2482, .T. ) ;
#45499=SURFACE_STYLE_FILL_AREA ( #95876 ) ;
#45500=CIRCLE ( 'NONE', #9973, 0.1000000000000002554 ) ;
#45501=EDGE_CURVE ( 'NONE', #31560, #47494, #51817, .T. ) ;
#45502=AXIS2_PLACEMENT_3D ( 'NONE', #11379, #2194, #32979 ) ;
#45503=CARTESIAN_POINT ( 'NONE',  ( 6.249999999999967137, 2.500000000000000000, 6.495190528383297135 ) ) ;
#45504=EDGE_CURVE ( 'NONE', #61083, #1993, #91516, .T. ) ;
#45505=EDGE_LOOP ( 'NONE', ( #32616, #25892, #24240, #2222 ) ) ;
#45506=EDGE_LOOP ( 'NONE', ( #65147, #47945 ) ) ;
#45507=ORIENTED_EDGE ( 'NONE', *, *, #44377, .T. ) ;
#45509=CARTESIAN_POINT ( 'NONE',  ( 8.349999999999919709, 12.50000000000000000, -2.165063509461101710 ) ) ;
#45511=DIRECTION ( 'NONE',  ( -4.274815082592931898E-19, -0.9999939076577903929, -0.003490651415223739937 ) ) ;
#45512=VECTOR ( 'NONE', #99468, 1000.000000000000000 ) ;
#45513=CIRCLE ( 'NONE', #7827, 0.09999999999999982514 ) ;
#45514=FACE_OUTER_BOUND ( 'NONE', #25490, .T. ) ;
#45516=VERTEX_POINT ( 'NONE', #49481 ) ;
#45517=CARTESIAN_POINT ( 'NONE',  ( 21.24754738303297330, 0.7337760880902002292, -4.182111650399407132 ) ) ;
#45518=AXIS2_PLACEMENT_3D ( 'NONE', #18998, #58951, #106740 ) ;
#45519=ORIENTED_EDGE ( 'NONE', *, *, #89578, .F. ) ;
#45520=CIRCLE ( 'NONE', #110538, 0.1000000000000002554 ) ;
#45521=CARTESIAN_POINT ( 'NONE',  ( 11.44999999999990514, 2.500000000000000000, 2.611473670974873151 ) ) ;
#45522=FACE_OUTER_BOUND ( 'NONE', #108678, .T. ) ;
#45523=DIRECTION ( 'NONE',  ( -0.000000000000000000, 1.000000000000000000, -0.000000000000000000 ) ) ;
#45524=ORIENTED_EDGE ( 'NONE', *, *, #46331, .F. ) ;
#45525=DIRECTION ( 'NONE',  ( 0.000000000000000000, 0.000000000000000000, -1.000000000000000000 ) ) ;
#45526=CARTESIAN_POINT ( 'NONE',  ( -12.49999999999999467, 12.50000000000000000, 0.6277270498435161272 ) ) ;
#45527=AXIS2_PLACEMENT_3D ( 'NONE', #103074, #53343, #72974 ) ;
#45529=ORIENTED_EDGE ( 'NONE', *, *, #38213, .T. ) ;
#45530=AXIS2_PLACEMENT_3D ( 'NONE', #128793, #10282, #107834 ) ;
#45531=CARTESIAN_POINT ( 'NONE',  ( 10.84999999999991260, 2.500000000000000000, 6.495190528383297135 ) ) ;
#45532=ADVANCED_FACE ( 'NONE', ( #70391 ), #35096, .T. ) ;
#45533=AXIS2_PLACEMENT_3D ( 'NONE', #70320, #90588, #40881 ) ;
#45534=EDGE_LOOP ( 'NONE', ( #42240, #108933 ) ) ;
#45535=ORIENTED_EDGE ( 'NONE', *, *, #11883, .F. ) ;
#45536=CARTESIAN_POINT ( 'NONE',  ( 11.44999999999991047, 12.50000000000000000, -2.576566944158915184 ) ) ;
#45537=VECTOR ( 'NONE', #19841, 1000.000000000000000 ) ;
#45538=VERTEX_POINT ( 'NONE', #58003 ) ;
#45539=DIRECTION ( 'NONE',  ( -0.000000000000000000, 1.000000000000000000, -0.000000000000000000 ) ) ;
#45540=CARTESIAN_POINT ( 'NONE',  ( 11.04999999999990656, 2.500000000000000000, 2.611473670974873151 ) ) ;
#45541=CONICAL_SURFACE ( 'NONE', #41349, 0.1000000000000002554, 0.003490658503988666988 ) ;
#45542=DIRECTION ( 'NONE',  ( 0.000000000000000000, 0.000000000000000000, -1.000000000000000000 ) ) ;
#45543=EDGE_CURVE ( 'NONE', #40133, #105571, #129336, .T. ) ;
#45544=ORIENTED_EDGE ( 'NONE', *, *, #29329, .T. ) ;
#45545=CIRCLE ( 'NONE', #108226, 0.1000000000000002554 ) ;
#45546=FACE_BOUND ( 'NONE', #114843, .T. ) ;
#45547=CARTESIAN_POINT ( 'NONE',  ( 6.849999999999929479, 12.50000000000000000, -1.883746621131363597 ) ) ;
#45548=VERTEX_POINT ( 'NONE', #39029 ) ;
#45549=EDGE_CURVE ( 'NONE', #8757, #59390, #8234, .T. ) ;
#45550=CARTESIAN_POINT ( 'NONE',  ( -8.749999999999971578, 2.500000000000000000, 6.595190528383296780 ) ) ;
#45551=AXIS2_PLACEMENT_3D ( 'NONE', #13564, #25984, #85537 ) ;
#45552=DIRECTION ( 'NONE',  ( 0.000000000000000000, -0.9999939076577903929, 0.003490651415223739937 ) ) ;
#45553=EDGE_CURVE ( 'NONE', #107210, #18914, #33048, .T. ) ;
#45554=VERTEX_POINT ( 'NONE', #10186 ) ;
#45555=AXIS2_PLACEMENT_3D ( 'NONE', #89390, #67805, #118839 ) ;
#45556=EDGE_LOOP ( 'NONE', ( #57358, #29835, #105495, #97352 ) ) ;
#45557=ORIENTED_EDGE ( 'NONE', *, *, #118530, .F. ) ;
#45558=CARTESIAN_POINT ( 'NONE',  ( -0.8000000000000376810, 12.50000000000000000, -4.330127018922201643 ) ) ;
#45559=DIRECTION ( 'NONE',  ( 0.000000000000000000, 1.000000000000000000, 0.000000000000000000 ) ) ;
#45560=DIRECTION ( 'NONE',  ( -0.000000000000000000, 1.000000000000000000, -0.000000000000000000 ) ) ;
#45561=EDGE_CURVE ( 'NONE', #43214, #75247, #108374, .T. ) ;
#45562=FACE_BOUND ( 'NONE', #107307, .T. ) ;
#45563=ORIENTED_EDGE ( 'NONE', *, *, #15513, .T. ) ;
#45565=DIRECTION ( 'NONE',  ( 0.000000000000000000, -0.9999939076577903929, 0.003490651415223739937 ) ) ;
#45566=DIRECTION ( 'NONE',  ( 0.000000000000000000, 0.000000000000000000, 1.000000000000000000 ) ) ;
#45567=DIRECTION ( 'NONE',  ( 0.000000000000000000, 1.000000000000000000, -0.000000000000000000 ) ) ;
#45568=DIRECTION ( 'NONE',  ( 1.000000000000000000, 0.000000000000000000, 0.000000000000000000 ) ) ;
#45569=LINE ( 'NONE', #94642, #126287 ) ;
#45570=DIRECTION ( 'NONE',  ( 0.000000000000000000, 0.000000000000000000, 1.000000000000000000 ) ) ;
#45572=DIRECTION ( 'NONE',  ( 0.000000000000000000, 0.000000000000000000, 1.000000000000000000 ) ) ;
#45573=EDGE_LOOP ( 'NONE', ( #108170, #71407, #22604, #722 ) ) ;
#45574=ORIENTED_EDGE ( 'NONE', *, *, #42146, .T. ) ;
#45575=ORIENTED_EDGE ( 'NONE', *, *, #89777, .T. ) ;
#45576=ORIENTED_EDGE ( 'NONE', *, *, #46746, .F. ) ;
#45577=ORIENTED_EDGE ( 'NONE', *, *, #83843, .T. ) ;
#45578=DIRECTION ( 'NONE',  ( 0.000000000000000000, 1.000000000000000000, 0.000000000000000000 ) ) ;
#45579=DIRECTION ( 'NONE',  ( 0.000000000000000000, 0.000000000000000000, 1.000000000000000000 ) ) ;
#45580=EDGE_LOOP ( 'NONE', ( #42985, #53183 ) ) ;
#45581=FACE_BOUND ( 'NONE', #58031, .T. ) ;
#45582=DIRECTION ( 'NONE',  ( 0.000000000000000000, 0.000000000000000000, -1.000000000000000000 ) ) ;
#45583=AXIS2_PLACEMENT_3D ( 'NONE', #91824, #41456, #13239 ) ;
#45584=ADVANCED_FACE ( 'NONE', ( #78295 ), #50125, .T. ) ;
#45585=AXIS2_PLACEMENT_3D ( 'NONE', #121820, #81883, #73365 ) ;
#45586=DIRECTION ( 'NONE',  ( 0.000000000000000000, 0.000000000000000000, 1.000000000000000000 ) ) ;
#45587=ORIENTED_EDGE ( 'NONE', *, *, #116890, .T. ) ;
#45588=CARTESIAN_POINT ( 'NONE',  ( 8.549999999999918998, 12.50000000000000000, -1.883746621131363597 ) ) ;
#45589=CARTESIAN_POINT ( 'NONE',  ( -6.650000000000019007, 12.50000000000000000, -1.407149913249512663 ) ) ;
#45590=EDGE_CURVE ( 'NONE', #20424, #79817, #18347, .T. ) ;
#45591=DIRECTION ( 'NONE',  ( 0.000000000000000000, 0.000000000000000000, 1.000000000000000000 ) ) ;
#45592=ORIENTED_EDGE ( 'NONE', *, *, #20772, .T. ) ;
#45594=CIRCLE ( 'NONE', #116582, 0.06509327318403745899 ) ;
#45595=ADVANCED_FACE ( 'NONE', ( #88741 ), #5811, .T. ) ;
#45596=ORIENTED_EDGE ( 'NONE', *, *, #112679, .F. ) ;
#45597=CIRCLE ( 'NONE', #39354, 0.06509327318403745899 ) ;
#45598=ORIENTED_EDGE ( 'NONE', *, *, #117527, .F. ) ;
#45599=ORIENTED_EDGE ( 'NONE', *, *, #80366, .T. ) ;
#45600=ADVANCED_FACE ( 'NONE', ( #118199 ), #99845, .T. ) ;
#45601=DIRECTION ( 'NONE',  ( -4.274815082592931898E-19, -0.9999939076577903929, -0.003490651415223739937 ) ) ;
#45602=DIRECTION ( 'NONE',  ( 0.000000000000000000, 0.000000000000000000, 1.000000000000000000 ) ) ;
#45603=EDGE_CURVE ( 'NONE', #73436, #38247, #78937, .T. ) ;
#45604=DIRECTION ( 'NONE',  ( 0.000000000000000000, 1.000000000000000000, 0.000000000000000000 ) ) ;
#45605=EDGE_CURVE ( 'NONE', #79650, #102847, #124966, .T. ) ;
#45606=ORIENTED_EDGE ( 'NONE', *, *, #8063, .T. ) ;
#45607=CARTESIAN_POINT ( 'NONE',  ( 2.500000000000002220, 1.499999999999999556, -9.999999999999998224 ) ) ;
#45608=EDGE_CURVE ( 'NONE', #48547, #128936, #57773, .T. ) ;
#45609=CIRCLE ( 'NONE', #5763, 0.1000000000000002554 ) ;
#45610=DIRECTION ( 'NONE',  ( -0.000000000000000000, 1.000000000000000000, -0.000000000000000000 ) ) ;
#45611=CARTESIAN_POINT ( 'NONE',  ( 6.849999999999929479, 2.500000000000000000, -1.818653347947326138 ) ) ;
#45612=ADVANCED_FACE ( 'NONE', ( #95757 ), #20416, .T. ) ;
#45614=CARTESIAN_POINT ( 'NONE',  ( -0.4000000000000392131, 2.500000000000000000, -4.330127018922201643 ) ) ;
#45615=AXIS2_PLACEMENT_3D ( 'NONE', #98437, #99111, #76886 ) ;
#45616=DIRECTION ( 'NONE',  ( 0.000000000000000000, 1.000000000000000000, 0.000000000000000000 ) ) ;
#45617=ORIENTED_EDGE ( 'NONE', *, *, #59743, .T. ) ;
#45618=DIRECTION ( 'NONE',  ( -0.000000000000000000, 1.000000000000000000, -0.000000000000000000 ) ) ;
#45619=EDGE_CURVE ( 'NONE', #119267, #18141, #37496, .T. ) ;
#45620=CIRCLE ( 'NONE', #106154, 0.09999999999999982514 ) ;
#45621=ORIENTED_EDGE ( 'NONE', *, *, #70105, .T. ) ;
#45622=ORIENTED_EDGE ( 'NONE', *, *, #36899, .T. ) ;
#45623=CIRCLE ( 'NONE', #118765, 0.06509327318403745899 ) ;
#45624=CARTESIAN_POINT ( 'NONE',  ( 3.549999999999942979, 12.50000000000000000, 1.818653347947321475 ) ) ;
#45625=DIRECTION ( 'NONE',  ( 0.000000000000000000, 0.000000000000000000, -1.000000000000000000 ) ) ;
#45626=DIRECTION ( 'NONE',  ( 0.000000000000000000, -0.9999939076577903929, 0.003490651415223739937 ) ) ;
#45627=VECTOR ( 'NONE', #115450, 1000.000000000000000 ) ;
#45628=ORIENTED_EDGE ( 'NONE', *, *, #11140, .T. ) ;
#45629=AXIS2_PLACEMENT_3D ( 'NONE', #33401, #1336, #72032 ) ;
#45630=ORIENTED_EDGE ( 'NONE', *, *, #88516, .F. ) ;
#45631=DIRECTION ( 'NONE',  ( 0.000000000000000000, 0.000000000000000000, -1.000000000000000000 ) ) ;
#45632=CIRCLE ( 'NONE', #3847, 0.1000000000000000472 ) ;
#45633=CARTESIAN_POINT ( 'NONE',  ( 0.3999999999999563904, 2.500000000000000000, 4.922947341949748257 ) ) ;
#45634=CARTESIAN_POINT ( 'NONE',  ( 3.949999999999941558, 2.500000000000000000, -1.818653347947326138 ) ) ;
#45635=ORIENTED_EDGE ( 'NONE', *, *, #13818, .F. ) ;
#45636=ORIENTED_EDGE ( 'NONE', *, *, #5948, .F. ) ;
#45637=DIRECTION ( 'NONE',  ( 0.000000000000000000, -0.9999939076577903929, 0.003490651415223739937 ) ) ;
#45638=AXIS2_PLACEMENT_3D ( 'NONE', #114646, #106755, #37398 ) ;
#45639=ORIENTED_EDGE ( 'NONE', *, *, #27946, .T. ) ;
#45640=CARTESIAN_POINT ( 'NONE',  ( 0.5999999999999560130, 2.500000000000000000, -3.983716857408426293 ) ) ;
#45641=CARTESIAN_POINT ( 'NONE',  ( 7.099999999999927702, 12.50000000000000000, -3.702399969078687292 ) ) ;
#45642=ORIENTED_EDGE ( 'NONE', *, *, #61565, .T. ) ;
#45643=DIRECTION ( 'NONE',  ( 0.000000000000000000, -0.000000000000000000, 1.000000000000000000 ) ) ;
#45644=DIRECTION ( 'NONE',  ( 0.000000000000000000, 0.000000000000000000, 1.000000000000000000 ) ) ;
#45645=CARTESIAN_POINT ( 'NONE',  ( -3.470671598752761919E-14, 2.500000000000000000, -0.7928203230275518987 ) ) ;
#45646=CIRCLE ( 'NONE', #60323, 0.1000000000000002554 ) ;
#45647=DIRECTION ( 'NONE',  ( 0.000000000000000000, -0.9999939076577903929, 0.003490651415223739937 ) ) ;
#45648=ORIENTED_EDGE ( 'NONE', *, *, #50733, .T. ) ;
#45649=CARTESIAN_POINT ( 'NONE',  ( 13.34999999999990017, 12.50000000000000000, 1.472243186433545459 ) ) ;
#45650=AXIS2_PLACEMENT_3D ( 'NONE', #20420, #58425, #59722 ) ;
#45651=ADVANCED_FACE ( 'NONE', ( #38125 ), #8008, .T. ) ;
#45652=DIRECTION ( 'NONE',  ( -0.000000000000000000, -1.000000000000000000, -0.000000000000000000 ) ) ;
#45653=ORIENTED_EDGE ( 'NONE', *, *, #15812, .F. ) ;
#45654=ORIENTED_EDGE ( 'NONE', *, *, #121981, .F. ) ;
#45656=FACE_OUTER_BOUND ( 'NONE', #127324, .T. ) ;
#45657=DIRECTION ( 'NONE',  ( 0.000000000000000000, 0.000000000000000000, -1.000000000000000000 ) ) ;
#45658=CARTESIAN_POINT ( 'NONE',  ( 14.14999999999989377, 12.50000000000000000, -2.857883832488653741 ) ) ;
#45659=CARTESIAN_POINT ( 'NONE',  ( -7.100000000000013856, 2.500000000000000000, 3.537306695894645081 ) ) ;
#45660=CARTESIAN_POINT ( 'NONE',  ( 0.3999999999999568345, 2.500000000000000000, -5.122947341949753763 ) ) ;
#45661=EDGE_CURVE ( 'NONE', #47460, #63253, #76855, .T. ) ;
#45662=LINE ( 'NONE', #116306, #9357 ) ;
#45663=FACE_OUTER_BOUND ( 'NONE', #111902, .T. ) ;
#45664=DIRECTION ( 'NONE',  ( 0.000000000000000000, 0.000000000000000000, 1.000000000000000000 ) ) ;
#45665=CONICAL_SURFACE ( 'NONE', #110489, 0.1000000000000002554, 0.003490658503988666988 ) ;
#45667=EDGE_LOOP ( 'NONE', ( #46580, #126083, #29143, #30167 ) ) ;
#45668=CIRCLE ( 'NONE', #22687, 0.1000000000000002554 ) ;
#45669=VERTEX_POINT ( 'NONE', #125220 ) ;
#45670=CONICAL_SURFACE ( 'NONE', #28947, 0.1000000000000002554, 0.003490658503988666988 ) ;
#45671=VECTOR ( 'NONE', #92288, 1000.000000000000000 ) ;
#45672=ORIENTED_EDGE ( 'NONE', *, *, #107088, .T. ) ;
#45674=DIRECTION ( 'NONE',  ( 0.000000000000000000, 0.000000000000000000, 1.000000000000000000 ) ) ;
#45675=CIRCLE ( 'NONE', #14340, 0.06509327318403745899 ) ;
#45676=ORIENTED_EDGE ( 'NONE', *, *, #42193, .T. ) ;
#45677=AXIS2_PLACEMENT_3D ( 'NONE', #89733, #52385, #100204 ) ;
#45678=DIRECTION ( 'NONE',  ( -4.274815082592931898E-19, -0.9999939076577903929, -0.003490651415223739937 ) ) ;
#45679=CARTESIAN_POINT ( 'NONE',  ( 5.599999999999933031, 12.50000000000000000, -0.4115034346978157509 ) ) ;
#45680=CARTESIAN_POINT ( 'NONE',  ( -6.700000000000019718, 2.500000000000000000, -4.330127018922201643 ) ) ;
#45681=EDGE_LOOP ( 'NONE', ( #18471, #34499, #110836, #48185 ) ) ;
#45682=VECTOR ( 'NONE', #29937, 1000.000000000000000 ) ;
#45683=CARTESIAN_POINT ( 'NONE',  ( 2.899999999999944844, 12.50000000000000000, 3.572213422710607489 ) ) ;
#45684=ORIENTED_EDGE ( 'NONE', *, *, #103771, .F. ) ;
#45685=AXIS2_PLACEMENT_3D ( 'NONE', #94918, #95566, #15034 ) ;
#45686=EDGE_CURVE ( 'NONE', #71126, #121543, #46658, .T. ) ;
#45687=ORIENTED_EDGE ( 'NONE', *, *, #83463, .F. ) ;
#45688=ORIENTED_EDGE ( 'NONE', *, *, #122880, .T. ) ;
#45689=EDGE_LOOP ( 'NONE', ( #64846, #32937, #126014, #3682 ) ) ;
#45690=DIRECTION ( 'NONE',  ( -4.274815082592931898E-19, -0.9999939076577903929, -0.003490651415223739937 ) ) ;
#45691=LINE ( 'NONE', #85600, #63392 ) ;
#45692=DIRECTION ( 'NONE',  ( -0.000000000000000000, -1.000000000000000000, -0.000000000000000000 ) ) ;
#45693=DIRECTION ( 'NONE',  ( 0.000000000000000000, 0.000000000000000000, 1.000000000000000000 ) ) ;
#45694=CONICAL_SURFACE ( 'NONE', #118840, 0.09999999999999982514, 0.003490658503988666988 ) ;
#45695=EDGE_CURVE ( 'NONE', #42825, #100830, #49772, .T. ) ;
#45697=CLOSED_SHELL ( 'NONE', ( #13402, #81027, #87574, #20135, #119079, #52618, #70677, #102908, #45355, #41736, #92946, #119725, #43817, #93994, #1145, #39834, #11725, #55347, #128233, #74708, #94779, #44024, #20923, #91414, #32715, #72470, #98697, #21239, #119253, #85296, #21021, #87421, #78474, #121682, #12361, #23436, #76050, #61423, #5226, #41316, #32854, #51017, #39234, #111017, #15280, #128914, #91353, #57416, #100543, #80350, #21494, #87228, #57251, #38924, #129025, #125121, #79388, #69408, #9372, #19561, #124949, #123772, #119581, #41629, #107194, #32909, #24803, #4575, #4454, #21670, #125774, #65047, #88832, #100132, #50822, #61351, #44275, #115779, #4078, #124150, #100679, #51475, #93905, #74154, #18659, #46911, #91092, #50258, #103043, #21120, #23557, #13835, #8615, #69781, #5917, #45905, #58887, #124388, #61077, #123885, #86635, #124226, #56030, #45612, #111028, #11863, #92516, #104228, #31965, #17820, #27953, #59471, #30500, #18945, #22166, #115242, #31738, #119746, #22100, #41731, #100168, #109307, #50321, #54862, #74616, #90158, #105647, #68626, #58731, #26850, #60530, #17326, #124066, #80762, #50917, #51789, #65196, #103147, #33277, #82672, #98762, #403, #68893, #126913, #82043, #125664, #46276, #72928, #107542, #65104, #56347, #77499, #99420, #61713, #39271, #21518, #97538, #36150, #122555, #120490, #83460, #7951, #76720, #19430, #10276, #70213, #126804, #101861, #10422, #37469, #111650, #34328, #90930, #109692, #72225, #104810, #65422, #78681, #107321, #22267, #56489, #121364, #44969, #56641, #64335, #7316, #22936, #114873, #55362, #69617, #119472, #22513, #75600, #29961, #13177, #112575, #40585, #42447, #53772, #5936, #4565, #105112, #73027, #51543, #30395, #91014, #24760, #73205, #67905, #64725, #81796, #51918, #86798, #35280, #101708, #118607, #13771, #92287, #711, #35588, #22075, #16382, #42788, #4517, #59028, #16695, #120032, #122592, #89477, #101542, #58139, #25973, #45903, #113998, #3296, #104983, #127838, #14952, #120485, #2015, #80081, #17315, #129133, #20935, #129388, #72330, #39071, #118079, #52471, #109093, #114759, #128755, #61974, #76776, #38965, #65103, #118969, #74456, #117377, #37859, #28273, #62856, #89046, #65907, #22111, #113417, #51116, #38347, #109590, #53099, #78748, #109436, #39614, #10378, #27499, #81503, #27259, #6345, #50752, #8006, #37768, #78781, #115916, #4052, #102272, #13164, #13196, #125756, #17927, #118750, #71134, #48533, #120819, #57312, #111893, #56945, #36563, #58158, #42459, #109252, #71453, #36638, #103394, #57658, #99800, #20520, #81182, #925, #5983, #94602, #71400, #91726, #7258, #24585, #9534, #7360, #91094, #15009, #109750, #12029, #76304, #115033, #20399, #57980, #120357, #84675, #30956, #69032, #6006, #25612, #77924, #119599, #4386, #85738, #79560, #106724, #74098, #112036, #70230, #57095, #57726, #21505, #33631, #113454, #59539, #92557, #13094, #65255, #63435, #37038, #44870, #90761, #114756, #58763, #19736, #37271, #47950, #63340, #28700, #6437, #109242, #7303, #56228, #28015, #106265, #101703, #1707, #125215, #73046, #46564, #88210, #126059, #73756, #86946, #11872, #127020, #84607, #22734, #128831, #105838, #64588, #25125, #109665, #66224, #53255, #125988, #11257, #25370, #62411, #34963, #82668, #88583, #100255, #97692, #108093, #32298, #96638, #82084, #97754, #75143, #11299, #101223, #27430, #18866, #68157, #107520, #112835, #1116, #39158, #83937, #52755, #87263, #20412, #93054, #89871, #12318, #97133, #31780, #41625, #62879, #98799, #36727, #12610, #73818, #125829, #83608, #2273, #121218, #15888, #85791, #3022, #20057, #58632, #89372, #109243, #27359, #43344, #38889, #98290, #112433, #90618, #1220, #115107, #44764, #90183, #102890, #55617, #117344, #25175, #90906, #66275, #29744, #1895, #86624, #4315, #107417, #4140, #20575, #15854, #96691, #33470, #45045, #123473, #49125, #9808, #110209, #7470, #102030, #45442, #35396, #87725, #72472, #28604, #25634, #56784, #66100, #88785, #83394, #93205, #117061, #90712, #84899, #108269, #119428, #73356, #69085, #48356, #48314, #85173, #103946, #107145, #98168, #33079, #82407, #102827, #46020, #55200, #73802, #86377, #81374, #66526, #19374, #45600, #55351, #90012, #89881, #56438, #114237, #31283, #72329, #128070, #75278, #21585, #6357, #93220, #15220, #55523, #6296, #117307, #33885, #114152, #87907, #81516, #76143, #25816, #111175, #41626, #80917, #44656, #107463, #125788, #72067, #21106, #9529, #9332, #59481, #39221, #115269, #87781, #93794, #82498, #100548, #99621, #24169, #9745, #29231, #23920, #91098, #72888, #12662, #95677, #53826, #30707, #16503, #47247, #48683, #54651, #125275, #86169, #8721, #112929, #114858, #38858, #43433, #103051, #13924, #72167, #22830, #118444, #54458, #83565, #122351, #99822, #21612, #23734, #1807, #68562, #37570, #51777, #79694, #107354, #15434, #32657, #62719, #33074, #32449, #61991, #85485, #62149, #64377, #68633, #129394, #108579, #35835, #13456, #66510, #8883, #99575, #122301, #80610, #45129, #68097, #12602, #36991, #112972, #47164, #32408, #5678, #125218, #22210, #14071, #87676, #111065, #17379, #100246, #60421, #42620, #63173, #122835, #121645, #121070, #86689, #102440, #21027, #54163, #100295, #119518, #116030, #6647, #76756, #24718, #27136, #45008, #18323, #120089, #17388, #77655, #70049, #47632, #52826, #87685, #101597, #84890, #7669, #72231, #12374, #124230, #51391, #11581, #24586, #63120, #19937, #108509, #6532, #69088, #112376, #54041, #61361, #107383, #127525, #75864, #82717, #98764, #35677, #73654, #98573, #128808, #58170, #62232, #68059, #60345, #22242, #104237, #117630, #106566, #37066, #87084, #15771, #15997, #106252, #23860, #92136, #102712, #10985, #99088, #69736, #113554, #88221, #106880, #77090, #104281, #12923, #98194, #105487, #35110, #29804, #42998, #10864, #29323, #40260, #25163, #114086, #20813, #78077, #25650, #106563, #33889, #79303, #113979, #125811, #107565, #1643, #124781, #9393, #84542, #101756, #24280, #61399, #58058, #103856, #43695, #73878, #119698, #121856, #56179, #68265, #95981, #51971, #25729, #113255, #121619, #85069, #114977, #7418, #25287, #23982, #72465, #33331, #3745, #73363, #37578, #118821, #84911, #71622, #109257, #74107, #31216, #123116, #33776, #75197, #62758, #74843, #59526, #28763, #7160, #128489, #47977, #14645, #113252, #76770, #52212, #30728, #33013, #54380, #113895, #46109, #91251, #32005, #127175, #105077, #115476, #10521, #23971, #63530, #20296, #37625, #17335, #97861, #60008, #119138, #62135, #129387, #87193, #4299, #37220, #54593, #60501, #69824, #36419, #52570, #60196, #66568, #49130, #53935, #50310, #14708, #79574, #70012, #108577, #92251, #129120, #93926, #121978, #23269, #76821, #22237, #14085, #53266, #127894, #97020, #92588, #86301, #8424, #101769, #107190, #108611, #32932, #118981, #117621, #47543, #108626, #59700, #83997, #30233, #31388, #43236, #14800, #4963, #18032, #121776, #103859, #54047, #103672, #75546, #61249, #3485, #40870, #59373, #12930, #91975, #43417, #77343, #119734, #23818, #6826, #100084, #81495, #80882, #106055, #47080, #124489, #32463, #62874, #109305, #83945, #116017, #18611, #77341, #48120, #84604, #37158, #102575, #57898, #114535, #34569, #23321, #116016, #67735, #21340, #81085, #57987, #62558, #33596, #42928, #28333, #124224, #19887, #15177, #85045, #40741, #110573, #119129, #56180, #36831, #14791, #11673, #120183, #125841, #17216, #70272, #37588, #7750, #7462, #930, #48051, #66196, #10826, #36532, #6943, #82683, #45865, #108425, #1938, #33383, #14006, #50156, #125116, #34796, #98685, #79305, #100858, #33327, #11867, #22847, #55013, #16319, #71289, #127060, #71098, #116755, #24905, #42613, #83469, #87976, #47794, #6538, #85875, #67173, #86036, #128335, #21502, #45595, #35417, #8459, #126599, #21175, #100550, #95467, #34977, #125536, #99673, #49292, #115924, #5572, #116448, #7321, #127375, #81958, #36585, #641, #43728, #83979, #24443, #94197, #97396, #121691, #45703, #50575, #77743, #29318, #104070, #65019, #15873, #92151, #94643, #74261, #1432, #60209, #69345, #84794, #73338, #11748, #29977, #48059, #61813, #82666, #24912, #103014, #2736, #3651, #39100, #77911, #75039, #123373, #101133, #33287, #78422, #117957, #70862, #16448, #107618, #2866, #105698, #100148, #114790, #52830, #75151, #85928, #32610, #22595, #65938, #759, #81334, #2536, #82657, #3140, #43674, #92340, #12022, #46072, #49595, #50043, #87966, #112675, #68039, #108051, #40926, #104926, #128680, #124384, #10222, #23552, #11475, #56959, #20705, #86044, #126860, #6093, #69458, #107743, #45285, #47658, #75428, #102867, #17257, #111136, #85048, #89931, #91834, #37113, #51486, #56738, #29966, #38698, #107962, #56337, #43837, #125610, #102487, #24493, #121681, #112191, #17224, #36823, #60206, #103389, #36600, #114724, #15693, #122021, #7310, #75543, #124604, #478, #2573, #41050, #80472, #9795, #41482, #26072, #86676, #50369, #46659, #61392, #34389, #64437, #28911, #109747, #65192, #59368, #111222, #66529, #92031, #23817, #60806, #124665, #121461, #21676, #56320, #51947, #24292, #112820, #34071, #19877, #101813, #102851, #12138, #63760, #7792, #49190, #34054, #101702, #44120, #72883, #14710, #109824, #86475, #48702, #15449, #33473, #22561, #37612, #27684, #92238, #99918, #75140, #124555, #97931, #27118, #114437, #71444, #127584, #42072, #39551, #78823, #110018, #115492, #87096, #124945, #86998, #114908, #108682, #105909, #74273, #103385, #14949, #27523, #25333, #4013, #100535, #129373, #41723, #28685, #24958, #109365, #63442, #94592, #84256, #108480, #7531, #48964, #125780, #31086, #39588, #118688, #103794, #78584, #115144, #92675, #74424, #6663, #15388, #123002, #53994, #88012, #4783, #65190, #77539, #68307, #60452, #100841, #32393, #54004, #21959, #69512, #89791, #109140, #33590, #49346, #127626, #82235, #108927, #97231, #128275, #116583, #4208, #94943, #6640, #30051, #34640, #4215, #105029, #103289, #35525, #67685, #80766, #70122, #118869, #120178, #52268, #67004, #42091, #98429, #100705, #95254, #62163, #25554, #108986, #33772, #11730, #46931, #91672, #93565, #26218, #92712, #30669, #126429, #8785, #13311, #104224, #176, #24439, #118330, #89797, #34469, #56424, #57392, #34537, #41882, #105285, #59951, #107951, #48966, #113519, #109150, #37776, #111501, #123315, #44500, #33228, #69796, #62630, #106489, #14855, #27209, #16105, #47808, #17488, #18639, #91513, #115097, #123587, #107044, #54405, #74713, #10012, #93412, #105338, #33824, #60262, #81414, #37317, #22090, #30744, #63022, #2133, #81698, #10105, #16020, #71585, #80570, #71747, #89993, #90683, #125984, #96965, #46360, #60913, #82225, #66832, #110153, #103954, #105365, #29352, #89647, #46299, #4068, #88236, #70261, #58716, #125360, #57682, #82053, #52362, #48214, #5422, #70829, #1496, #107096, #80179, #123423, #104935, #127734, #116385, #94289, #17748, #119179, #114213, #121110, #72010, #127726, #2175, #35206, #23091, #100849, #103612, #64460, #115601, #97192, #17601, #102962, #101601, #1391, #42684, #16839, #87041, #93302, #129127, #20037, #66284, #120130, #53474, #63769, #91924, #27165, #66017, #54981, #99609, #66982, #10569, #77812, #90175, #32299, #21824, #70680, #15880, #104546, #64165, #24440, #11147, #101580, #95506, #118176, #40296, #33182, #21826, #71495, #47056, #38486, #37154, #97011, #117677, #103643, #54467, #89221, #89149, #106857, #60110, #81896, #13593, #79796, #42516, #96549, #76580, #33004, #26692, #36331, #69852, #56256, #9526, #23264, #114693, #78692, #12181, #10107, #75189, #103962, #72314, #75985, #94869, #54451, #2137, #6249, #30651, #27469, #71162, #93105, #63909, #102753, #53566, #11550, #94930, #33673, #72230, #16675, #39592, #338, #47375, #49277, #93042, #111444, #33634, #68804, #76918, #66372, #43066, #84913, #34797, #89322, #5327, #3268, #102637, #108673, #55296, #123479, #29343, #87047, #91690, #92313, #100833, #61828, #73486, #38692, #61294, #37871, #3613, #2280, #49279, #122966, #88733, #283, #106577, #127031, #58422, #94323, #62998, #9365, #12510, #95737, #91518, #37584, #85734, #13355, #27213, #59260, #128258, #80605, #111560, #57420, #108516, #81544, #112455, #31275, #109847, #116395, #83990, #18926, #29015, #64740, #101259, #98929, #15910, #52119, #112416, #29969, #105091, #14944, #48786, #107938, #51247, #62566, #61877, #35692, #6654, #75982, #80776, #79869, #110461, #114291, #15065, #4203, #44115, #41054, #65046, #8481, #22191, #118298, #47325, #76407, #64901, #10511, #104589, #116411, #93452, #115468, #6565, #35170, #31074, #55574, #33578, #2672, #103805, #77203, #31679, #128238, #77049, #86517, #78841, #22086, #65962, #113879, #5213, #73253, #5729, #32760, #41099, #113410, #39555, #85634, #113892, #113082, #81894, #57513, #74970, #78255, #112218, #36735, #114700, #21852, #103396, #45080, #91111, #88882, #96585, #54355, #122125, #120217, #44693, #87991, #30829, #20132, #88287, #119763, #32923, #128164, #94599, #30825, #85216, #38356, #3525, #64203, #43182, #74069, #50408, #27580, #26974, #111900, #69565, #60661, #7572, #64500, #76283, #113125, #29421, #117353, #1543, #37920, #49870, #119712, #62969, #3335, #48540, #59086, #56242, #36270, #118117, #25076, #108912, #106822, #5267, #120804, #1234, #14704, #118065, #49714, #39889, #57404, #23282, #27845, #18663, #126168, #11985, #110554, #51200, #61728, #28163, #1855, #52104, #18065, #5512, #65371, #95667, #40428, #17981, #90731, #68790, #46738, #90774, #37861, #118020, #484, #67724, #121966, #87208, #40906, #80009, #11820, #2689, #114289, #22682, #63613, #118141, #121780, #29902, #15168, #110454, #85638, #85459, #30998, #42021, #82195, #108277, #12178, #67897, #116600, #119033, #69150, #120904, #100894, #11777, #42457, #106571, #74943, #53894, #10169, #49955, #100292, #65587, #57900, #11254, #23679, #110834, #17627, #10700, #6348, #59810, #46075, #94436, #101126, #4903, #60671, #6832, #127170, #122191, #99470, #119928, #117192, #74975, #79232, #6870, #102348, #41039, #72728, #35405, #84159, #91677, #46032, #18570, #22103, #98581, #89591, #94835, #89557, #31597, #62619, #126856, #93354, #110570, #100129, #76455, #44537, #78849, #90494, #56185, #94294, #71726, #75919, #118842, #4201, #98316, #123910, #109845, #63969, #93398, #114655, #17819, #44967, #103533, #38649, #7464, #38183, #61397, #87819, #47404, #106474, #32562, #39996, #125037, #56958, #115029, #109095, #30798, #38978, #123121, #62404, #12198, #88323, #120238, #74113, #27408, #110293, #34046, #70516, #9322, #84092, #62913, #3031, #96432, #73932, #123645, #19109, #129068, #42889, #78415, #6110, #113561, #8450, #7195, #119016, #58561, #47757, #75713, #27388, #73048, #30130, #125835, #86247, #79312, #53851, #65194, #129546, #48275, #80885, #87, #44918, #120344, #70994, #35354, #127791, #81234, #111455, #82990, #19612, #17283, #62302, #124011, #18981, #96676, #70598, #77183, #125376, #93864, #121015, #128487, #63277, #108822, #31688, #101441, #81588, #72935, #26210, #99507, #17036, #22034, #54009, #81637, #65527, #70671, #51841, #117786, #51567, #56582, #113237, #71581, #54595, #77449, #110471, #49987, #78353, #23600, #97037, #9175, #87341, #9234, #62394, #120707, #27015, #124547, #7155, #15290, #102891, #111459, #112685, #30987, #122594, #99027, #90288, #11143, #31129, #125715, #125624, #7135, #91576, #70724, #41153, #44388, #127286, #17, #1076, #111004, #51959, #94691, #54214, #95259, #74658, #42735, #29236, #66819, #23374, #18070, #108378, #29480, #16736, #71920, #96550, #47797, #33569, #15708, #102185, #66589, #88072, #114923, #27354, #61131, #80733, #20607, #60432, #57224, #7481, #128212, #70726, #84433, #59809, #128614, #126695, #57118, #113614, #68462, #48370, #67266, #84998, #39493, #115117, #110474, #32538, #124054, #118030, #51384, #52338, #94354, #93287, #69364, #106020, #68474, #95978, #22718, #23364, #29578, #43792, #40824, #7483, #86692, #98165, #24907, #85076, #63780, #28746, #59883, #51494, #1581, #61661, #76134, #73047, #74334, #665, #21297, #110313, #318, #8931, #72779, #114592, #29652, #95512, #115208, #78248, #34369, #57073, #118720, #53952, #13012, #60535, #102340, #108265, #10430, #75711, #53897, #3131, #92395, #52685, #35426, #97784, #97138, #56348, #124014, #88219, #89165, #26228, #34886, #84499, #58455, #72784, #35783, #55748, #32277, #10231, #79922, #25971, #116762, #93316, #51554, #95458, #37205, #30068, #45311, #91240, #28651, #34212, #60095, #63959, #129221, #97964, #58143, #30345, #78565, #61778, #28001, #119685, #10804, #18819, #106069, #77402, #9193, #33881, #121128, #34532, #31386, #128337, #31847, #93121, #98072, #89778, #72680, #6408, #119532, #23539, #29326, #127412, #5695, #70763, #57666, #43251, #88848, #24328, #75455, #11228, #75248, #40730, #4563, #107026, #99686, #73339, #18826, #116328, #72160, #66999, #11556, #26942, #65679, #24028, #27866, #27572, #70102, #123432, #44215, #108125, #58309, #26323, #28123, #7731, #90677, #89614, #71301, #19835, #37436, #45651, #1874, #67879, #30552, #43566, #71439, #120674, #108810, #47700, #49184, #42792, #32705, #116913, #90603, #104065, #123067, #93626, #28546, #5115, #17325, #44130, #61742, #125459, #60818, #50909, #81171, #125131, #102911, #119277, #20307, #35106, #36090, #92237, #47958, #2105, #89879, #106221, #22107, #94058, #107183, #39542, #68392, #69189, #81505, #83690, #110152, #125364, #93425, #7988, #80399, #43055, #88377, #94827, #105850, #57734, #114443, #25735, #1252, #80974, #7890, #121394, #99964, #16291, #85783, #40040, #17312, #72367, #19723, #78956, #21484, #78149, #59044, #78739, #49044, #29919, #128823, #63433, #52814, #18136, #66110, #85726, #41412, #123679, #71525, #18563, #12779, #4304, #77856, #112787, #88234, #4614, #47641, #81744, #58301, #80281, #119123, #25581, #99294, #23433, #82952, #56505, #101648, #111779, #63599, #27512, #26394, #91536, #116693, #64371, #10714, #34535, #18350, #101296, #82058, #83233, #87359, #66122, #30080, #55051, #11472, #108985, #23534, #112524, #5473, #97649, #111268, #8930, #58931, #7421, #49422, #9539, #110611, #71051, #106473, #53839, #27696, #59053, #112488, #62456, #94332, #74249, #29608, #28345, #77635, #66664, #15540, #12693, #82574, #103240, #65134, #56506, #128511, #69508, #36166, #7397, #51483, #38191, #14198, #86866, #90441, #17245, #43605, #79043, #105589, #109136, #62723, #61237, #7156, #84272, #122702, #80478, #121953, #68608, #51397, #58211, #21063, #33014, #122689, #77189, #120286, #18354, #29914, #118270, #89407, #38529, #69344, #79321, #83701, #112098, #75869, #3907, #89925, #42096, #76147, #111992, #94587, #83703, #69205, #28769, #76197, #102646, #85156, #9832, #17810, #50118, #127630, #70412, #67754, #28447, #2112, #38375, #89294, #108361, #113363, #4465, #36882, #84690, #69102, #31224, #58161, #35013, #65619, #106369, #17063, #42134, #72281, #92283, #50571, #97244, #28844, #2791, #26392, #60777, #25214, #125052, #94600, #60482, #107884, #46035, #54548, #57453, #106162, #47653, #34935, #22776, #105099, #21074, #20380, #83294, #376, #124291, #108249, #75538, #110714, #93309, #82408, #17680, #7152, #13085, #3614, #67289, #122296, #50225, #61574, #111517, #104667, #41492, #104119, #60768, #45028, #69526, #42844, #2880, #128042, #87680, #3776, #127104, #73552, #26799, #9614, #49699, #112629, #96523, #71239, #35420, #103347, #33000, #10099, #92460, #48075, #10271, #4145, #65224, #64988, #115760, #27244, #6154, #80622, #89281, #8474, #107040, #127336, #69673, #88070, #75396, #47550, #53726, #101663, #53149, #106686, #38045, #101147, #84412, #109789, #28927, #46631, #122543, #2372, #104517, #66746, #42288, #126540, #84849, #63901, #122714, #110770, #3992, #8027, #14503, #126996, #32614, #100451, #36000, #108470, #7707, #91856, #83798, #114384, #123724, #52667, #43834, #77462, #108040, #2115, #63667, #99571, #26537, #50631, #62466, #70462, #113230, #29950, #98628, #93001, #6823, #9952, #51641, #45146, #104046, #112100, #7654, #78985, #89630, #1397, #76208, #33126, #126476, #37146, #6108, #9158, #80454, #71141, #98639, #106995, #5506, #102036, #42668, #128235, #129552, #11131, #94753, #101750, #73343, #18407, #73649, #67006, #117443, #74357, #50739, #754, #75243, #1711, #8323, #41369, #6931, #68843, #82344, #30967, #129132, #60375, #109433, #63508, #66431, #86899, #17439, #1063, #128500, #74663, #96067, #45346, #37322, #42469, #69357, #47556, #28159, #28571, #76664, #117113, #96208, #84645, #69958, #50737, #30397, #78675, #82959, #104522, #77094, #69808, #35424, #93549, #95237, #51399, #6725, #17206, #16018, #14643, #47483, #49602, #40855, #116956, #6239, #14755, #60360, #91735, #21559, #106807, #53264, #36695, #8567, #61220, #32915, #98587, #25733, #44216, #41359, #86800, #53718, #42674, #79917, #74257, #51342, #57014, #102500, #28750, #101302, #3591, #99097, #51642, #31633, #124743, #51378, #119910, #110450, #88527, #19901, #83138, #82393, #23429, #76712, #128344, #122482, #31704, #72623, #112192, #116329, #62869, #95421, #78663, #3705, #95576, #43646, #127430, #38971, #123874, #21880, #15436, #77493, #31438, #37516, #64644, #94032, #122679, #93238, #81801, #108208, #105741, #113103, #47786, #122017, #5939, #56517, #31834, #60611, #56244, #26801, #22154, #50467, #87983, #114707, #43356, #26793, #60963, #107301, #114293, #4154, #52265, #124155, #12402, #69349, #79255, #10372, #24496, #74761, #14394, #56975, #110881, #112532, #32014, #86050, #49854, #30924, #35129, #125654, #85569, #127135, #43553, #99796, #63664, #96808, #8831, #16440, #71019, #83830, #657, #39842, #29194, #85103, #42528, #117806, #34691, #127426, #69971, #42520, #128154, #5166, #85587, #77120, #108620, #12764, #77799, #114914, #18714, #53167, #43663, #36271, #21675, #106053, #84694, #10969, #35520, #88601, #111793, #100398, #20292, #52374, #97350, #113893, #9687, #63905, #91034, #113234, #35793, #70992, #104887, #56694, #473, #14327, #46629, #105007, #64531, #86464, #91520, #82516, #9028, #30862, #108520, #25064, #123732, #13606, #68529, #78068, #64777, #44961, #6233, #126958, #59848, #127180, #84311, #99812, #108730, #40843, #22988, #97286, #118926, #71788, #118227, #34049, #2825, #28450, #18000, #83698, #78060, #100936, #6163, #85944, #26700, #91987, #82405, #32903, #28282, #108836, #67144, #106615, #40900, #35972, #34216, #87399, #125228, #56018, #39062, #84268, #31952, #92301, #100020, #118852, #380, #91787, #15206, #31829, #22716, #110410, #81363, #54205, #124391, #87356, #86778, #51800, #37155, #114578, #52272, #40090, #41727, #60157, #27674, #49755, #68312, #45225, #64957, #56909, #28712, #20714, #44701, #47172, #22882, #78626, #53722, #59819, #22932, #81096, #117060, #76765, #99009, #91990, #28798, #31209, #104272, #25868, #95266, #48126, #3769, #112674, #10071, #20343, #116313, #8, #46322, #63226, #107360, #40230, #73332, #21768, #14940, #86673, #120496, #55630, #44474, #12149, #2992, #63516, #61092, #124638, #8210, #90666, #53095, #83151, #61826, #79682, #83549, #56183, #27965, #18863, #61992, #128926, #108795, #88415, #108676, #116486, #7518, #13175, #13252, #120657, #69, #106471, #37932, #89456, #97215, #104374, #13501, #71755, #56245, #81015, #29585, #74510, #111329, #33054, #96221, #73916, #92471, #3730, #90936, #43560, #107483, #69776, #82722, #105855, #46754, #37770, #30904, #10931, #81492, #20466, #66736, #127577, #15420, #32911, #9319, #120298, #70219, #123979, #106715, #18285, #27996, #103977, #95819, #18247, #1438, #61930, #72936, #5847, #96743, #124488, #77032, #29097, #54455, #26382, #42954, #82329, #71894, #10672, #39288, #89899, #10461, #60517, #128971, #88409, #76483, #12747, #28919, #16760, #58681, #6662, #100840, #42439, #102132, #26899, #38973, #108375, #59651, #21814, #70513, #62345, #113400, #81238, #81092, #11999, #62548, #68453, #34945, #82340, #83757, #104114, #17703, #20606, #108962, #18967, #11891, #89422, #4722, #8407, #55199, #6100, #93796, #121112, #62773, #41525, #53098, #29564, #43358, #40245, #97916, #35019, #100396, #125383, #94036, #68309, #42503, #10555, #30031, #2886, #29495, #40298, #53684, #18399, #10924, #129512, #75604, #71127, #99256, #98427, #81811, #26340, #117035, #37465, #96993, #9698, #87250, #49266, #69849, #60964, #29538, #117858, #66374, #104105, #9949, #75392, #122459, #41430, #105084, #80825, #6091, #3597, #87582, #13759, #15233, #84173, #40597, #86016, #47065, #52407, #90332, #38364, #56193, #36575, #59961, #73104, #14075, #74162, #106708, #32340, #32628, #8776, #8773, #37032, #40671, #93027, #93732, #76040, #128771, #59527, #89924, #27159, #24172, #92409, #102021, #61081, #82913, #91189, #43685, #116952, #99991, #33338, #76719, #109203, #92913, #81582, #120401, #67500, #47489, #104672, #89889, #33466, #94986, #57918, #116346, #124107, #1077, #66088, #103379, #122917, #43991, #34706, #3339, #104436, #100769, #89376, #87458, #38956, #74668, #87670, #114713, #41458, #1067, #97294, #77082, #73829, #50419, #44650, #21345, #23116, #46652, #27492, #15870, #19574, #97592, #46465, #40986, #69629, #113457, #100619, #111471, #68577, #115312, #43658, #21067, #50187, #115010, #127219, #8758, #34637, #55716, #38795, #83958, #17821, #6991, #64078, #102119, #89037, #25021, #25362, #49702, #121791, #78004, #111166, #41110, #28010, #80575, #121396, #9866, #79861, #42910, #123282, #24014, #6644, #39708, #10751, #105753, #83661, #64488, #33087, #127354, #111030, #127572, #96220, #18240, #119753, #51030, #36741, #94396, #107203, #82288, #45768, #120017, #49132, #15866, #36579, #5220, #26662, #89139, #2740, #92662, #113250, #112986, #86937, #69833, #67272, #100785, #16431, #49215, #114132, #27357, #91085, #104206, #116476, #77244, #45899, #98748, #41831, #51410, #72488, #43923, #28484, #36421, #24605, #72173, #34276, #118421, #51069, #31378, #9106, #52112, #11242, #120077, #19416, #80722, #29801, #16799, #120073, #36794, #98906, #3039, #91209, #105269, #86921, #80182, #101236, #126448, #72872, #49710, #15430, #127466, #66846, #22993, #93056, #55674, #123338, #34755, #84536, #79236, #94047, #87102, #89214, #26958, #8879, #113982, #66889, #117102, #24137, #4831, #5779, #31971, #124168, #47640, #118759, #105097, #81281, #17049, #120236, #46153, #121231, #115008, #106641, #126594, #92843, #34645, #125390, #50188, #41306, #97298, #126115, #46121, #114670, #38384, #84824, #35944, #129297, #15687, #32120, #38102, #80073, #22659, #14257, #10737, #60353, #13339, #126762, #56294, #96967, #1644, #105481, #53975, #54980, #45760, #102017, #24342, #788, #74840, #22427, #107260, #32697, #116649, #43420, #18551, #90330, #79094, #121248, #124049, #6064, #53833, #60378, #59295, #61860, #69103, #76297, #35265, #68959, #21007, #96286, #60635, #81600, #47815, #66268, #52485, #95984, #62612, #122143, #83034, #111387, #72340, #125937, #80615, #103655, #66775, #39985, #128393, #24454, #27509, #101442, #73341, #1851, #1960, #89043, #42948, #4729, #31698, #97610, #63011, #27864, #81793, #57571, #93621, #119701, #119809, #8157, #30827, #29438, #66697, #19740, #11000, #33782, #126998, #70503, #111280, #77972, #21982, #74827, #107689, #35247, #79416, #14235, #85340, #59150, #38544, #90506, #46269, #593, #69679, #108206, #81017, #116331, #33639, #80774, #312, #55374, #57244, #123024, #82808, #7848, #7574, #125042, #71380, #121738, #18446, #67937, #80296, #70750, #26881, #21321, #65510, #110726, #78426, #64527, #51585, #125375, #9537, #13654, #88666, #57126, #32003, #114135, #90024, #113722, #52257, #111371, #1135, #126032, #18090, #12035, #43256, #91729, #52261, #66989, #106145, #94178, #55157, #19734, #87722, #3446, #120583, #68218, #47469, #109316, #48700, #22983, #64950, #41571, #42628, #103338, #112547, #93157, #69041, #57652, #105044, #94336, #84993, #15113, #111231, #109909, #54322, #108757, #49142, #33225, #109407, #106166, #51951, #106588, #75447, #117626, #60324, #74828, #125331, #101298, #125508, #100798, #99417, #87669, #115720, #35359, #92900, #74307, #37641, #53665, #10042, #38527, #18662, #49289, #41490, #25206, #49129, #116499, #22974, #20716, #69683, #71961, #93207, #7835, #81910, #37307, #22397, #17333, #14557, #66787, #68470, #78357, #120193, #102335, #119270, #88721, #12050, #74309, #24131, #1859, #1343, #88694, #116964, #123266, #44305, #48081, #27401, #31375, #77309, #82167, #105293, #10956, #28320, #74551, #104582, #74573, #33239, #38094, #2531, #105264, #68722, #27121, #108193, #79353, #14056, #89828, #106637, #70270, #23554, #106736, #76605, #47645, #81510, #50799, #14653, #12518, #113379, #44825, #78999, #41397, #32866, #90432, #122619, #91419, #89739, #86030, #128677, #102077, #11736, #85003, #55465, #105853, #22956, #71409, #73308, #8217, #62807, #33340, #74564, #65020, #129381, #85219, #120232, #42344, #97341, #117471, #35545, #53274, #88078, #24020, #32294, #91940, #89329, #40746, #45532, #73130, #13299, #58715, #101854, #118923, #27961, #7153, #66627, #21765, #5627, #49655, #29082, #86783, #97435, #28335, #95826, #56063, #25306, #2008, #99249, #47954, #75717, #83116, #123181, #19746, #99133, #40505, #121685, #129201, #26181, #103159, #30701, #118340, #88213, #27664, #119861, #107786, #51815, #39938, #54855, #53916, #392, #77194, #1974, #66971, #14491, #21511, #96227, #11781, #6492, #4451, #6000, #100792, #70813, #20179, #119595, #17814, #33231, #108965, #60361, #94185, #21840, #23717, #19283, #10417, #104074, #67825, #31039, #85683, #93876, #25822, #114195, #81731, #24230, #14559, #30954, #11413, #106179, #42334, #31846, #125679, #127013, #128569, #23110, #107481, #56349, #10005, #68051, #82937, #79244, #13073, #37056, #3172, #40310, #91587, #27267, #63024, #75300, #119199, #105161, #94929, #88402, #22794, #16848, #71801, #4460, #88570, #11994, #126530, #115158, #36940, #12439, #81047, #77647, #85158, #82289, #27066, #24338, #47390, #109235, #125562, #10008, #114588, #53984, #107745, #114400, #120977, #65357, #88589, #28913, #120242, #125230, #12130, #27737, #9054, #10057, #45131, #3925, #120644, #25628, #68185, #31522, #127747, #112091, #112772, #25172, #126537, #84705, #113508, #89527, #87668, #62601, #115470, #86785, #6258, #48796, #124003, #86720, #43665, #8461, #119642, #102651, #81318, #27257, #61136, #54165, #56911, #122872, #109378, #109583, #2579, #8767, #85476, #117905, #38634, #57886, #81574, #21188, #52256, #36788, #46772, #61816, #91685, #104017, #25795, #94491, #49273, #19114, #129233, #120090, #31511, #74260, #44561, #26647, #15802, #124801, #90451, #116637, #77581, #81250, #121363, #112360, #92719, #116177, #62711, #97872, #62675, #13241, #102617, #97761, #20293, #104468, #62614, #127121, #29285, #11162, #104126, #124235, #90988, #55164, #33715, #105393, #22253, #27789, #106109, #96869, #67453, #56550, #124695, #87195, #102490, #113090, #53200, #29903, #117536, #101760, #75640, #34717, #78731, #102382, #4153, #97556, #100530, #79705, #33903, #57989, #5604, #40480, #56247, #125663, #74849, #59018, #116656, #127174, #21926, #129484, #90028, #43963, #58884, #23486, #92727, #55632, #71748, #58625, #4110, #11751, #88994, #17879, #108340, #105426, #85789, #127428, #3898, #82817, #94484, #126588, #99665, #20463, #126077, #81089, #122389, #62429, #19377, #31998, #9678, #44850, #95364, #107686, #21348, #72474, #122131, #115319, #54154, #59693, #92893, #123407, #83541, #58719, #129234, #55207, #101922, #26960, #29181, #61552, #75233, #45770, #86213, #81944, #44255, #103278, #104832, #83397, #85965, #70988, #17381, #129066, #52501, #5038, #28864, #25811, #104678, #70263, #95350, #115058, #114722, #108146, #119341, #123270, #107644, #6213, #73457, #54762, #107798, #6205, #102004, #53178, #53574, #84451, #24275, #55564, #47078, #24692, #78836, #61619, #70846, #15120, #11086, #27625, #121839, #76566, #37168, #17111, #20623, #80036, #11571, #69674, #48863, #84155, #75386, #99032, #44461, #122156, #227, #55214, #76629, #96491, #122995, #101118, #114136, #47395, #33614, #54159, #117117, #43530, #67740, #45811, #41711, #38622, #125619, #90038, #13244, #62192, #88337, #41207, #65524, #120065, #59312, #116855, #120985, #107317, #2683, #123176, #37477, #65365, #4472, #83717, #87094, #99556, #123571, #48254, #81938, #68007, #99356, #89008, #12634, #49393, #108316, #55024, #107839, #115165, #54136, #53413, #127259, #43740, #56339, #85935, #72000, #10808, #44752, #88233, #28067, #79964, #24757, #69640, #18728, #41644, #77486, #85882, #48544, #86520, #76703, #17055, #71731, #39854, #74203, #59388, #63816, #117503, #26400, #127028, #53332, #87867, #11529, #48202, #117846, #63101, #51908, #32061, #9046, #5522, #85149, #14942, #35821, #21958, #3752, #80937, #35534, #12859, #125214, #105677, #1363, #91602, #68046, #15823, #28382, #101183, #29617, #124746, #65215, #95525, #104540, #48071, #15549, #112988, #70422, #94208, #115328, #53716, #55453, #75823, #37324, #117944, #79455, #19560, #97998, #33865, #49140, #31799, #56657, #52216, #57835, #124347, #118603, #81623, #92731, #106622, #75718, #80865, #100503, #68488, #128819, #41986, #14938, #27734, #33638, #112365, #39119, #73215, #105737, #20854, #36733, #62096, #4220, #52821, #23268, #91429, #55923, #63159, #35724, #45286, #56907, #126450, #2751, #609, #79459, #67946, #80498, #55610, #113829, #117351, #104720, #16110, #43583, #42946, #44704, #39536, #8256, #49443, #42795, #30813, #84145, #49544, #42873, #59485, #5155, #83929, #9035, #58633, #125385, #53593, #17153, #126092, #213, #84600, #36843, #11154, #124216, #56003, #435, #70377, #4730, #118487, #79770, #80444, #58718, #34214, #57880, #43667, #43969, #4445, #41300, #73667, #36093, #121857, #26851, #46367, #41937, #105889, #97018, #17765, #96263, #61254, #64020, #19625, #111951, #75, #15564, #93556, #38416, #126828, #22828, #82009, #98760, #2218, #23411, #115157, #13806, #76364, #118705, #96089, #43188, #127827, #10176, #103706, #60678, #47026, #24399, #114458, #127321, #113144, #77907, #75252, #18956, #30196, #72108, #10652, #39701, #21490, #43405, #129404, #85374, #67384, #31369, #122142, #30186, #98912, #128816, #108301, #48877, #70166, #90686, #3082, #105905, #118133, #34379, #68045, #120768, #73212, #125931, #125618, #106318, #73837, #25177, #81591, #69058, #19121, #8311, #15644, #21083, #120494, #98462, #44214, #109848, #6660, #90682, #58783, #16728, #83983, #114377, #7143, #31278, #96510, #6697, #17657, #87812, #17342, #45952, #75800, #81878, #77782, #127419, #79195, #38881, #42188, #34696, #74513, #9791, #96132, #34792, #91398, #63444, #18814, #1959, #50481, #15451, #18185, #129248, #120639, #105435, #92737, #30097, #74106, #19061, #25429, #59082, #82022, #126268, #35608, #14396, #127315, #45584, #8302, #23217, #94449, #65891, #39417, #57262, #85466, #104267, #20824, #107781, #14244, #97594, #129412, #72953, #56402, #87790, #96623, #1790, #96794, #61972, #78311, #75290, #50896, #74723, #12612, #23450, #93736, #50716, #89721, #66165, #6813, #105147, #54923, #54146, #16491, #107491, #83386, #117, #94389, #106572, #107647, #59689, #103229, #36992, #122297, #93892, #77866, #1721, #41260, #59653, #92303, #92135, #63705, #30699, #94487, #67074, #1241, #36577, #117229, #63131, #6243, #27667, #113573, #7570, #34868, #64049, #74572, #116169, #38461, #31619, #80929, #108494, #10562, #36486, #18084, #35372, #71437, #55787, #108979, #84947, #112511, #40087, #3288, #12309, #1388, #95563, #88752, #119422, #15667, #26703, #15374, #27018, #102733, #28544, #35879, #13660, #79550, #52042, #59582, #89065, #44818, #127227, #123716, #1404, #57123, #71711, #102952, #55408, #54103, #79701, #103895, #30246, #97706, #119438, #68833, #39110, #33343, #59817, #59614, #46901, #95247, #103793, #116217, #66732, #38669, #117691, #32188, #126742, #29027, #12771, #120597, #79822, #68943, #75094, #104665, #106408, #26856, #5854, #15231, #102894, #90513, #58869, #57946, #96377, #122457, #8160, #71571, #118719, #114440, #125606, #97450, #36072, #42615, #61138, #71002, #113832, #62417, #81917, #128396, #63169, #122602, #115608, #88471, #39703, #29338, #90444, #37677, #129447, #16589, #73937, #102748, #19062, #16836, #52361, #90777, #30324, #55356, #122095, #90203, #65039, #93632, #115491, #65777, #113967, #107467, #94182, #115161, #77628, #7875, #107836, #81266, #122445, #90526, #121961, #125164, #94201, #24070, #34240, #123849, #65113, #22504, #34378, #84319, #17611, #28453, #17487, #2408, #113551, #22972, #57669, #117267, #95529, #105263, #6094, #128610, #113725, #101924, #85114, #68937, #21827, #51484, #123727, #10947, #49193, #70371, #126871, #120505, #84056, #116233, #52531, #51061, #31136, #57064, #98014, #4881, #7903, #7408, #89169, #68323, #87087, #14720, #33763, #63585, #37001, #107244, #120240, #54611, #106625, #101065, #102628, #40543, #93718, #3912, #61236, #56630, #126357, #124906, #59781, #21289, #22159, #75399, #120699, #21844, #114349, #73465, #92241, #78200, #965, #118915, #54620, #22416, #10710, #121519, #28261, #30383, #49434, #31961, #1194, #51066, #30814, #99523, #46750, #8719, #15726, #48845, #126848, #68792, #95687, #93786, #127656, #22567, #45864, #33988, #85478, #83281, #88303, #78677, #9644, #79608, #66958, #32929, #59143, #62919, #43843, #73203, #90084, #15262, #64423, #62563, #110921, #23438, #63661, #115105, #96859, #67580, #25270, #14956, #82652, #122443, #52529, #109934, #64570, #110885, #107221, #39444, #17506, #46841, #85833, #122397, #14476, #112104, #61568, #20458, #9850, #79951, #6104, #89309, #127877, #87147, #6817, #71389, #106719, #7423, #918, #23275, #45451, #89010, #34371, #112888, #66254, #78418, #23595, #102797, #129347, #44224, #112990, #70591, #33731, #99512, #20727, #94012, #102919, #114921, #69338, #107305, #38168, #18705, #107928 ) ) ;
#45698=DIRECTION ( 'NONE',  ( -4.274815082592931898E-19, -0.9999939076577903929, -0.003490651415223739937 ) ) ;
#45699=EDGE_LOOP ( 'NONE', ( #32168, #95297, #104246, #20127 ) ) ;
#45700=CIRCLE ( 'NONE', #127182, 0.06509327318403745899 ) ;
#45701=CARTESIAN_POINT ( 'NONE',  ( -11.44999999999999751, 2.500000000000000000, -2.411473670974874306 ) ) ;
#45702=CARTESIAN_POINT ( 'NONE',  ( -5.000000000000024869, 2.500000000000000000, -4.922947341949753586 ) ) ;
#45703=ADVANCED_FACE ( 'NONE', ( #117961 ), #112460, .T. ) ;
#45704=CARTESIAN_POINT ( 'NONE',  ( -4.400000000000028777, 2.500000000000000000, -4.776537180435978414 ) ) ;
#45705=CARTESIAN_POINT ( 'NONE',  ( 19.40342015654640306, -2.551666867760341795, 4.359384978532470534 ) ) ;
#45706=EDGE_CURVE ( 'NONE', #87575, #84331, #27022, .T. ) ;
#45707=ORIENTED_EDGE ( 'NONE', *, *, #114284, .T. ) ;
#45708=VERTEX_POINT ( 'NONE', #108144 ) ;
#45710=ORIENTED_EDGE ( 'NONE', *, *, #56214, .F. ) ;
#45711=DIRECTION ( 'NONE',  ( 0.000000000000000000, 0.000000000000000000, -1.000000000000000000 ) ) ;
#45712=DIRECTION ( 'NONE',  ( 0.000000000000000000, 0.000000000000000000, 1.000000000000000000 ) ) ;
#45713=DIRECTION ( 'NONE',  ( 0.000000000000000000, 1.000000000000000000, 0.000000000000000000 ) ) ;
#45714=EDGE_CURVE ( 'NONE', #102404, #63670, #25718, .T. ) ;
#45715=FACE_BOUND ( 'NONE', #33300, .T. ) ;
#45716=CARTESIAN_POINT ( 'NONE',  ( 14.34999999999989662, 2.500000000000000000, 2.611473670974873151 ) ) ;
#45717=CARTESIAN_POINT ( 'NONE',  ( -10.84999999999999964, 12.50000000000000000, 1.472243186433545459 ) ) ;
#45718=AXIS2_PLACEMENT_3D ( 'NONE', #105347, #125611, #26146 ) ;
#45719=DIRECTION ( 'NONE',  ( 0.000000000000000000, -0.9999939076577903929, 0.003490651415223739937 ) ) ;
#45720=DIRECTION ( 'NONE',  ( 0.000000000000000000, 0.000000000000000000, 1.000000000000000000 ) ) ;
#45721=AXIS2_PLACEMENT_3D ( 'NONE', #87696, #67380, #96218 ) ;
#45723=DIRECTION ( 'NONE',  ( 0.000000000000000000, 1.000000000000000000, 0.000000000000000000 ) ) ;
#45724=CONICAL_SURFACE ( 'NONE', #62454, 0.1000000000000002554, 0.003490658503988666988 ) ;
#45725=DIRECTION ( 'NONE',  ( 0.000000000000000000, 1.000000000000000000, 0.000000000000000000 ) ) ;
#45726=DIRECTION ( 'NONE',  ( -0.000000000000000000, -1.000000000000000000, -0.000000000000000000 ) ) ;
#45727=AXIS2_PLACEMENT_3D ( 'NONE', #90272, #121680, #10442 ) ;
#45728=ORIENTED_EDGE ( 'NONE', *, *, #12566, .F. ) ;
#45729=ORIENTED_EDGE ( 'NONE', *, *, #110141, .F. ) ;
#45730=ORIENTED_EDGE ( 'NONE', *, *, #27831, .T. ) ;
#45731=ORIENTED_EDGE ( 'NONE', *, *, #108659, .F. ) ;
#45732=CONICAL_SURFACE ( 'NONE', #39491, 0.1000000000000002554, 0.003490658503988666988 ) ;
#45733=CARTESIAN_POINT ( 'NONE',  ( -7.100000000000017408, 12.50000000000000000, -3.637306695894650055 ) ) ;
#45734=FACE_BOUND ( 'NONE', #41971, .T. ) ;
#45735=CARTESIAN_POINT ( 'NONE',  ( 14.99999999999992895, 2.500000000000000000, -2.276824562219559311E-15 ) ) ;
#45736=VECTOR ( 'NONE', #72310, 1000.000000000000000 ) ;
#45737=VECTOR ( 'NONE', #8324, 1000.000000000000000 ) ;
#45738=EDGE_LOOP ( 'NONE', ( #11256, #94544 ) ) ;
#45739=CARTESIAN_POINT ( 'NONE',  ( 7.899999999999923084, 2.500000000000000000, -0.6928203230275542523 ) ) ;
#45740=CARTESIAN_POINT ( 'NONE',  ( 8.099999999999923261, 12.50000000000000000, 3.983716857408420076 ) ) ;
#45741=ORIENTED_EDGE ( 'NONE', *, *, #67624, .T. ) ;
#45742=PLANE ( 'NONE',  #74115 ) ;
#45743=CARTESIAN_POINT ( 'NONE',  ( 1.649999999999948841, 2.500000000000000000, 6.395190528383296602 ) ) ;
#45744=EDGE_CURVE ( 'NONE', #98189, #17267, #16270, .T. ) ;
#45746=AXIS2_PLACEMENT_3D ( 'NONE', #66013, #75824, #5783 ) ;
#45747=EDGE_CURVE ( 'NONE', #51306, #79214, #53867, .T. ) ;
#45748=CARTESIAN_POINT ( 'NONE',  ( -4.600000000000024514, 2.500000000000000000, 0.6928203230275494784 ) ) ;
#45749=CARTESIAN_POINT ( 'NONE',  ( 4.349999999999936584, 12.50000000000000000, 6.083687093685482772 ) ) ;
#45750=EDGE_CURVE ( 'NONE', #59076, #22957, #70590, .T. ) ;
#45751=EDGE_CURVE ( 'NONE', #99163, #96734, #104038, .T. ) ;
#45752=EDGE_LOOP ( 'NONE', ( #109768, #6566 ) ) ;
#45753=AXIS2_PLACEMENT_3D ( 'NONE', #97505, #49070, #127612 ) ;
#45754=CARTESIAN_POINT ( 'NONE',  ( -4.800000000000022915, 2.500000000000000000, 4.083716857408420609 ) ) ;
#45755=AXIS2_PLACEMENT_3D ( 'NONE', #65753, #28429, #55305 ) ;
#45756=CARTESIAN_POINT ( 'NONE',  ( -13.09999999999999254, 2.500000000000000000, -3.883716857408423984 ) ) ;
#45757=ORIENTED_EDGE ( 'NONE', *, *, #26237, .F. ) ;
#45758=CIRCLE ( 'NONE', #24820, 0.06509327318403745899 ) ;
#45759=DIRECTION ( 'NONE',  ( -0.000000000000000000, -1.000000000000000000, -0.000000000000000000 ) ) ;
#45760=ADVANCED_FACE ( 'NONE', ( #106844 ), #58078, .T. ) ;
#45761=VERTEX_POINT ( 'NONE', #15893 ) ;
#45762=VERTEX_POINT ( 'NONE', #46025 ) ;
#45763=CARTESIAN_POINT ( 'NONE',  ( 0.1999999999999571565, 2.500000000000000000, 3.983716857408420076 ) ) ;
#45764=CIRCLE ( 'NONE', #20719, 0.06509327318403745899 ) ;
#45765=ORIENTED_EDGE ( 'NONE', *, *, #97619, .F. ) ;
#45766=DIRECTION ( 'NONE',  ( 0.000000000000000000, 1.000000000000000000, 0.000000000000000000 ) ) ;
#45767=CARTESIAN_POINT ( 'NONE',  ( 2.899999999999946620, 12.50000000000000000, -0.6928203230275542523 ) ) ;
#45768=ADVANCED_FACE ( 'NONE', ( #85914 ), #125846, .T. ) ;
#45769=VECTOR ( 'NONE', #105183, 1000.000000000000000 ) ;
#45770=ADVANCED_FACE ( 'NONE', ( #68863 ), #93662, .T. ) ;
#45771=ORIENTED_EDGE ( 'NONE', *, *, #115310, .T. ) ;
#45772=CARTESIAN_POINT ( 'NONE',  ( 10.64999999999991331, 12.50000000000000000, 6.213873640053559022 ) ) ;
#45773=DIRECTION ( 'NONE',  ( -0.000000000000000000, -1.000000000000000000, -0.000000000000000000 ) ) ;
#45774=FACE_OUTER_BOUND ( 'NONE', #31502, .T. ) ;
#45775=DIRECTION ( 'NONE',  ( 0.000000000000000000, -0.000000000000000000, 1.000000000000000000 ) ) ;
#45776=CARTESIAN_POINT ( 'NONE',  ( -5.400000000000023448, 2.500000000000000000, -5.122947341949753763 ) ) ;
#45777=DIRECTION ( 'NONE',  ( -0.000000000000000000, -1.000000000000000000, -0.000000000000000000 ) ) ;
#45778=EDGE_CURVE ( 'NONE', #17717, #41136, #95809, .T. ) ;
#45779=AXIS2_PLACEMENT_3D ( 'NONE', #55996, #113642, #6237 ) ;
#45780=VERTEX_POINT ( 'NONE', #110085 ) ;
#45781=CONICAL_SURFACE ( 'NONE', #20731, 0.1000000000000002554, 0.003490658503988666988 ) ;
#45782=ORIENTED_EDGE ( 'NONE', *, *, #46870, .F. ) ;
#45783=DIRECTION ( 'NONE',  ( -0.000000000000000000, -1.000000000000000000, -0.000000000000000000 ) ) ;
#45784=CARTESIAN_POINT ( 'NONE',  ( 4.199999999999939782, 2.500000000000000000, -2.276824562219559311E-15 ) ) ;
#45785=DIRECTION ( 'NONE',  ( -0.000000000000000000, -1.000000000000000000, -0.000000000000000000 ) ) ;
#45786=EDGE_LOOP ( 'NONE', ( #56664, #117918 ) ) ;
#45787=VERTEX_POINT ( 'NONE', #48593 ) ;
#45788=ORIENTED_EDGE ( 'NONE', *, *, #96526, .F. ) ;
#45789=DIRECTION ( 'NONE',  ( 0.000000000000000000, 0.000000000000000000, -1.000000000000000000 ) ) ;
#45790=AXIS2_PLACEMENT_3D ( 'NONE', #98693, #10946, #110463 ) ;
#45791=DIRECTION ( 'NONE',  ( 0.7336674352945157240, 0.000000000000000000, 0.6795087154616692438 ) ) ;
#45793=DIRECTION ( 'NONE',  ( 0.000000000000000000, 0.000000000000000000, 1.000000000000000000 ) ) ;
#45794=DIRECTION ( 'NONE',  ( 0.000000000000000000, 0.000000000000000000, 1.000000000000000000 ) ) ;
#45796=CARTESIAN_POINT ( 'NONE',  ( -1.050000000000037348, 2.500000000000000000, -2.611473670974877592 ) ) ;
#45797=CONICAL_SURFACE ( 'NONE', #60382, 0.1000000000000002554, 0.003490658503988666988 ) ;
#45798=DIRECTION ( 'NONE',  ( 0.000000000000000000, 0.000000000000000000, -1.000000000000000000 ) ) ;
#45799=DIRECTION ( 'NONE',  ( 0.000000000000000000, 0.000000000000000000, 1.000000000000000000 ) ) ;
#45800=ORIENTED_EDGE ( 'NONE', *, *, #54545, .T. ) ;
#45801=VECTOR ( 'NONE', #109046, 1000.000000000000000 ) ;
#45802=DIRECTION ( 'NONE',  ( -0.000000000000000000, -1.000000000000000000, -0.000000000000000000 ) ) ;
#45803=EDGE_LOOP ( 'NONE', ( #120624, #91579 ) ) ;
#45804=ORIENTED_EDGE ( 'NONE', *, *, #41465, .T. ) ;
#45805=CARTESIAN_POINT ( 'NONE',  ( 8.949999999999919353, 12.50000000000000000, 2.511473670974873507 ) ) ;
#45806=DIRECTION ( 'NONE',  ( -0.000000000000000000, 1.000000000000000000, -0.000000000000000000 ) ) ;
#45807=CIRCLE ( 'NONE', #114740, 0.1000000000000002554 ) ;
#45808=CARTESIAN_POINT ( 'NONE',  ( -10.60000000000000142, 12.50000000000000000, 4.611443907251934426 ) ) ;
#45809=CARTESIAN_POINT ( 'NONE',  ( -3.150000000000029221, 2.500000000000000000, -1.718653347947326049 ) ) ;
#45810=CIRCLE ( 'NONE', #118957, 0.06509327318403745899 ) ;
#45811=ADVANCED_FACE ( 'NONE', ( #80637 ), #10132, .T. ) ;
#45812=CARTESIAN_POINT ( 'NONE',  ( 8.149999999999923972, 12.50000000000000000, 2.511473670974873507 ) ) ;
#45813=DIRECTION ( 'NONE',  ( -0.000000000000000000, 1.000000000000000000, -0.000000000000000000 ) ) ;
#45814=CARTESIAN_POINT ( 'NONE',  ( 10.39999999999991509, 12.50000000000000000, 0.7579135962115869374 ) ) ;
#45815=ORIENTED_EDGE ( 'NONE', *, *, #115000, .T. ) ;
#45816=FACE_OUTER_BOUND ( 'NONE', #85542, .T. ) ;
#45817=VECTOR ( 'NONE', #2282, 1000.000000000000000 ) ;
#45818=CARTESIAN_POINT ( 'NONE',  ( -3.749999999999994671, 2.500000000000000000, -6.495190528383302464 ) ) ;
#45819=ORIENTED_EDGE ( 'NONE', *, *, #111340, .F. ) ;
#45820=ORIENTED_EDGE ( 'NONE', *, *, #13506, .F. ) ;
#45821=AXIS2_PLACEMENT_3D ( 'NONE', #51788, #83185, #91707 ) ;
#45822=CIRCLE ( 'NONE', #73002, 0.06509327318403745899 ) ;
#45823=ORIENTED_EDGE ( 'NONE', *, *, #78213, .T. ) ;
#45824=AXIS2_PLACEMENT_3D ( 'NONE', #71657, #21928, #91946 ) ;
#45825=ORIENTED_EDGE ( 'NONE', *, *, #8443, .T. ) ;
#45826=LINE ( 'NONE', #115839, #125 ) ;
#45827=FACE_OUTER_BOUND ( 'NONE', #18599, .T. ) ;
#45828=CONICAL_SURFACE ( 'NONE', #18626, 0.1000000000000002554, 0.003490658503988666988 ) ;
#45829=CIRCLE ( 'NONE', #31173, 0.06509327318403745899 ) ;
#45830=FACE_OUTER_BOUND ( 'NONE', #125261, .T. ) ;
#45831=DIRECTION ( 'NONE',  ( 0.000000000000000000, -0.9999939076577903929, 0.003490651415223739937 ) ) ;
#45832=PLANE ( 'NONE',  #124468 ) ;
#45833=ORIENTED_EDGE ( 'NONE', *, *, #58558, .F. ) ;
#45834=CARTESIAN_POINT ( 'NONE',  ( -9.550000000000006040, 12.50000000000000000, -2.165063509461101710 ) ) ;
#45835=FACE_OUTER_BOUND ( 'NONE', #96972, .T. ) ;
#45836=VERTEX_POINT ( 'NONE', #21049 ) ;
#45837=EDGE_LOOP ( 'NONE', ( #100980, #90903, #20129, #17320 ) ) ;
#45838=ORIENTED_EDGE ( 'NONE', *, *, #32445, .T. ) ;
#45839=AXIS2_PLACEMENT_3D ( 'NONE', #108834, #109496, #99687 ) ;
#45840=CARTESIAN_POINT ( 'NONE',  ( -13.74999999999995381, 2.500000000000000000, 2.165063509461101265 ) ) ;
#45842=CARTESIAN_POINT ( 'NONE',  ( -5.200000000000022382, 2.500000000000000000, 4.676537180435972552 ) ) ;
#45843=VECTOR ( 'NONE', #105881, 1000.000000000000000 ) ;
#45845=ORIENTED_EDGE ( 'NONE', *, *, #92621, .F. ) ;
#45846=CARTESIAN_POINT ( 'NONE',  ( 1.049999999999954525, 2.500000000000000000, 1.818653347947321475 ) ) ;
#45847=FACE_OUTER_BOUND ( 'NONE', #69066, .T. ) ;
#45848=EDGE_CURVE ( 'NONE', #18914, #107210, #118789, .T. ) ;
#45849=CARTESIAN_POINT ( 'NONE',  ( -10.85000000000000142, 2.500000000000000000, -7.088010851410849966 ) ) ;
#45851=CARTESIAN_POINT ( 'NONE',  ( 4.149999999999941735, 12.50000000000000000, -5.737276932171712751 ) ) ;
#45852=EDGE_CURVE ( 'NONE', #13448, #63527, #98976, .T. ) ;
#45853=CONICAL_SURFACE ( 'NONE', #18745, 0.1000000000000002554, 0.003490658503988666988 ) ;
#45854=VERTEX_POINT ( 'NONE', #110718 ) ;
#45855=CIRCLE ( 'NONE', #18651, 0.06509327318403745899 ) ;
#45856=FACE_OUTER_BOUND ( 'NONE', #32803, .T. ) ;
#45857=ORIENTED_EDGE ( 'NONE', *, *, #96702, .F. ) ;
#45858=EDGE_CURVE ( 'NONE', #50154, #117751, #70674, .T. ) ;
#45859=EDGE_CURVE ( 'NONE', #50793, #33187, #116639, .T. ) ;
#45860=ORIENTED_EDGE ( 'NONE', *, *, #110866, .F. ) ;
#45861=ORIENTED_EDGE ( 'NONE', *, *, #128399, .T. ) ;
#45862=EDGE_CURVE ( 'NONE', #103702, #55739, #60366, .T. ) ;
#45863=DIRECTION ( 'NONE',  ( 0.000000000000000000, 0.000000000000000000, 1.000000000000000000 ) ) ;
#45864=ADVANCED_FACE ( 'NONE', ( #38800 ), #88499, .T. ) ;
#45865=ADVANCED_FACE ( 'NONE', ( #79976 ), #26854, .T. ) ;
#45866=FACE_BOUND ( 'NONE', #17567, .T. ) ;
#45867=CIRCLE ( 'NONE', #83435, 0.06509327318403745899 ) ;
#45869=DIRECTION ( 'NONE',  ( 0.000000000000000000, 0.000000000000000000, 1.000000000000000000 ) ) ;
#45870=CARTESIAN_POINT ( 'NONE',  ( 1.249999999999986899, 2.500000000000000000, 6.395190528383296602 ) ) ;
#45871=AXIS2_PLACEMENT_3D ( 'NONE', #128606, #1549, #99767 ) ;
#45872=AXIS2_PLACEMENT_3D ( 'NONE', #59066, #58430, #97053 ) ;
#45873=ORIENTED_EDGE ( 'NONE', *, *, #18812, .T. ) ;
#45874=DIRECTION ( 'NONE',  ( -0.000000000000000000, -1.000000000000000000, -0.000000000000000000 ) ) ;
#45876=EDGE_CURVE ( 'NONE', #87229, #124, #121188, .T. ) ;
#45877=DIRECTION ( 'NONE',  ( -0.000000000000000000, -1.000000000000000000, -0.000000000000000000 ) ) ;
#45878=DIRECTION ( 'NONE',  ( -0.000000000000000000, -1.000000000000000000, -0.000000000000000000 ) ) ;
#45879=ORIENTED_EDGE ( 'NONE', *, *, #90285, .F. ) ;
#45880=DIRECTION ( 'NONE',  ( -0.000000000000000000, 1.000000000000000000, -0.000000000000000000 ) ) ;
#45881=CARTESIAN_POINT ( 'NONE',  ( 1.449999999999952660, 2.500000000000000000, -6.841600689897078702 ) ) ;
#45882=AXIS2_PLACEMENT_3D ( 'NONE', #17905, #116110, #86651 ) ;
#45883=VERTEX_POINT ( 'NONE', #89796 ) ;
#45884=CARTESIAN_POINT ( 'NONE',  ( 11.44999999999990692, 12.50000000000000000, 1.883746621131358934 ) ) ;
#45885=FACE_BOUND ( 'NONE', #110637, .T. ) ;
#45886=CARTESIAN_POINT ( 'NONE',  ( 13.54999999999989768, 12.50000000000000000, -2.576566944158915184 ) ) ;
#45889=CARTESIAN_POINT ( 'NONE',  ( -1.850000000000033840, 2.500000000000000000, 2.511473670974873507 ) ) ;
#45890=ORIENTED_EDGE ( 'NONE', *, *, #38640, .T. ) ;
#45891=VERTEX_POINT ( 'NONE', #50509 ) ;
#45893=AXIS2_PLACEMENT_3D ( 'NONE', #62388, #13904, #33571 ) ;
#45894=VERTEX_POINT ( 'NONE', #59058 ) ;
#45897=CARTESIAN_POINT ( 'NONE',  ( 0.3999999999999559464, 2.500000000000000000, -4.330127018922201643 ) ) ;
#45898=DIRECTION ( 'NONE',  ( 0.000000000000000000, 0.000000000000000000, -1.000000000000000000 ) ) ;
#45899=ADVANCED_FACE ( 'NONE', ( #766 ), #60977, .T. ) ;
#45900=EDGE_CURVE ( 'NONE', #53553, #61962, #11225, .T. ) ;
#45901=FACE_OUTER_BOUND ( 'NONE', #84567, .T. ) ;
#45902=AXIS2_PLACEMENT_3D ( 'NONE', #120632, #119993, #21804 ) ;
#45903=ADVANCED_FACE ( 'NONE', ( #71429 ), #100018, .T. ) ;
#45904=ORIENTED_EDGE ( 'NONE', *, *, #21162, .F. ) ;
#45905=ADVANCED_FACE ( 'NONE', ( #49251 ), #127128, .T. ) ;
#45906=VERTEX_POINT ( 'NONE', #81898 ) ;
#45907=CARTESIAN_POINT ( 'NONE',  ( 7.499999999999925393, 2.500000000000000000, -3.637306695894650055 ) ) ;
#45908=CIRCLE ( 'NONE', #37507, 0.1000000000000002554 ) ;
#45909=CONICAL_SURFACE ( 'NONE', #16539, 0.09999999999999982514, 0.003490658503988666988 ) ;
#45910=DIRECTION ( 'NONE',  ( -0.000000000000000000, 1.000000000000000000, -0.000000000000000000 ) ) ;
#45911=PLANE ( 'NONE',  #5340 ) ;
#45912=DIRECTION ( 'NONE',  ( -0.000000000000000000, 1.000000000000000000, -0.000000000000000000 ) ) ;
#45913=AXIS2_PLACEMENT_3D ( 'NONE', #106904, #106272, #55248 ) ;
#45914=EDGE_LOOP ( 'NONE', ( #94994, #107625 ) ) ;
#45915=ORIENTED_EDGE ( 'NONE', *, *, #111782, .F. ) ;
#45916=FACE_BOUND ( 'NONE', #102595, .T. ) ;
#45917=EDGE_LOOP ( 'NONE', ( #49816, #16028, #24054, #122532 ) ) ;
#45918=EDGE_CURVE ( 'NONE', #40453, #22266, #42658, .T. ) ;
#45919=FACE_OUTER_BOUND ( 'NONE', #114275, .T. ) ;
#45920=DIRECTION ( 'NONE',  ( 0.000000000000000000, 0.000000000000000000, 1.000000000000000000 ) ) ;
#45921=EDGE_CURVE ( 'NONE', #5769, #78285, #62287, .T. ) ;
#45922=ORIENTED_EDGE ( 'NONE', *, *, #109842, .T. ) ;
#45923=DIRECTION ( 'NONE',  ( -0.000000000000000000, -1.000000000000000000, -0.000000000000000000 ) ) ;
#45924=AXIS2_PLACEMENT_3D ( 'NONE', #96032, #56721, #117573 ) ;
#45925=AXIS2_PLACEMENT_3D ( 'NONE', #47466, #70803, #102210 ) ;
#45926=CARTESIAN_POINT ( 'NONE',  ( -10.84999999999999964, 12.50000000000000000, 2.922977105672686982 ) ) ;
#45927=EDGE_CURVE ( 'NONE', #19851, #59088, #106275, .T. ) ;
#45928=CARTESIAN_POINT ( 'NONE',  ( -9.350000000000008527, 2.500000000000000000, -6.148780366869520897 ) ) ;
#45929=EDGE_CURVE ( 'NONE', #109646, #17565, #73371, .T. ) ;
#45930=PLANE ( 'NONE',  #103008 ) ;
#45931=DIRECTION ( 'NONE',  ( 0.000000000000000000, 0.000000000000000000, 1.000000000000000000 ) ) ;
#45932=DIRECTION ( 'NONE',  ( 0.000000000000000000, 0.000000000000000000, 1.000000000000000000 ) ) ;
#45934=FACE_OUTER_BOUND ( 'NONE', #65888, .T. ) ;
#45935=CARTESIAN_POINT ( 'NONE',  ( -1.850000000000033840, 2.500000000000000000, 6.048780366869521252 ) ) ;
#45936=EDGE_CURVE ( 'NONE', #35458, #111625, #60238, .T. ) ;
#45937=ORIENTED_EDGE ( 'NONE', *, *, #35533, .F. ) ;
#45938=ORIENTED_EDGE ( 'NONE', *, *, #113906, .T. ) ;
#45940=ORIENTED_EDGE ( 'NONE', *, *, #70567, .F. ) ;
#45941=CARTESIAN_POINT ( 'NONE',  ( -6.650000000000018119, 2.500000000000000000, -2.857883832488653741 ) ) ;
#45942=EDGE_LOOP ( 'NONE', ( #92782, #92072, #39757, #16650 ) ) ;
#45943=ORIENTED_EDGE ( 'NONE', *, *, #50963, .F. ) ;
#45944=ORIENTED_EDGE ( 'NONE', *, *, #69245, .F. ) ;
#45945=FACE_OUTER_BOUND ( 'NONE', #51357, .T. ) ;
#45946=AXIS2_PLACEMENT_3D ( 'NONE', #13954, #24431, #64351 ) ;
#45947=AXIS2_PLACEMENT_3D ( 'NONE', #88121, #78351, #116099 ) ;
#45949=CARTESIAN_POINT ( 'NONE',  ( 14.59999999999989484, 2.500000000000000000, 0.6928203230275494784 ) ) ;
#45950=DIRECTION ( 'NONE',  ( 0.000000000000000000, 1.000000000000000000, 0.000000000000000000 ) ) ;
#45952=ADVANCED_FACE ( 'NONE', ( #62917 ), #3982, .T. ) ;
#45953=ORIENTED_EDGE ( 'NONE', *, *, #20602, .F. ) ;
#45954=AXIS2_PLACEMENT_3D ( 'NONE', #28936, #49872, #88472 ) ;
#45955=AXIS2_PLACEMENT_3D ( 'NONE', #96492, #105699, #57230 ) ;
#45956=CARTESIAN_POINT ( 'NONE',  ( -11.04999999999999893, 12.50000000000000000, 6.083687093685482772 ) ) ;
#45957=CIRCLE ( 'NONE', #121155, 0.06509327318403745899 ) ;
#45958=ORIENTED_EDGE ( 'NONE', *, *, #14322, .F. ) ;
#45959=VERTEX_POINT ( 'NONE', #61640 ) ;
#45960=ORIENTED_EDGE ( 'NONE', *, *, #39285, .F. ) ;
#45961=VERTEX_POINT ( 'NONE', #54376 ) ;
#45962=CARTESIAN_POINT ( 'NONE',  ( 15.39999999999989200, 12.50000000000000000, -0.6928203230275542523 ) ) ;
#45963=VERTEX_POINT ( 'NONE', #112023 ) ;
#45964=VERTEX_POINT ( 'NONE', #93029 ) ;
#45965=AXIS2_PLACEMENT_3D ( 'NONE', #51845, #101583, #129136 ) ;
#45966=DIRECTION ( 'NONE',  ( 0.000000000000000000, -0.000000000000000000, 1.000000000000000000 ) ) ;
#45967=AXIS2_PLACEMENT_3D ( 'NONE', #35544, #76745, #57094 ) ;
#45968=DIRECTION ( 'NONE',  ( 0.000000000000000000, 1.000000000000000000, 0.000000000000000000 ) ) ;
#45969=DIRECTION ( 'NONE',  ( -0.000000000000000000, 1.000000000000000000, -0.000000000000000000 ) ) ;
#45970=VECTOR ( 'NONE', #101565, 1000.000000000000000 ) ;
#45971=EDGE_CURVE ( 'NONE', #104801, #124539, #120850, .T. ) ;
#45972=DIRECTION ( 'NONE',  ( 0.000000000000000000, 1.000000000000000000, 0.000000000000000000 ) ) ;
#45973=LINE ( 'NONE', #108735, #13625 ) ;
#45974=CARTESIAN_POINT ( 'NONE',  ( 1.849999999999949685, 12.50000000000000000, -2.446380397790840266 ) ) ;
#45975=ORIENTED_EDGE ( 'NONE', *, *, #33736, .T. ) ;
#45976=DIRECTION ( 'NONE',  ( -0.000000000000000000, -1.000000000000000000, -0.000000000000000000 ) ) ;
#45977=VECTOR ( 'NONE', #61639, 1000.000000000000000 ) ;
#45978=EDGE_LOOP ( 'NONE', ( #116881, #25657, #70684, #77115 ) ) ;
#45979=FACE_OUTER_BOUND ( 'NONE', #20175, .T. ) ;
#45980=ORIENTED_EDGE ( 'NONE', *, *, #110264, .F. ) ;
#45981=DIRECTION ( 'NONE',  ( 0.000000000000000000, 1.000000000000000000, 0.000000000000000000 ) ) ;
#45982=CONICAL_SURFACE ( 'NONE', #129533, 0.1000000000000000056, 0.003490658503988666988 ) ;
#45983=EDGE_LOOP ( 'NONE', ( #71209, #26044, #43977, #69118 ) ) ;
#45984=EDGE_CURVE ( 'NONE', #17050, #52727, #76939, .T. ) ;
#45985=EDGE_LOOP ( 'NONE', ( #72981, #71406 ) ) ;
#45986=DIRECTION ( 'NONE',  ( -0.000000000000000000, 1.000000000000000000, -0.000000000000000000 ) ) ;
#45987=DIRECTION ( 'NONE',  ( -0.000000000000000000, 1.000000000000000000, -0.000000000000000000 ) ) ;
#45989=FACE_OUTER_BOUND ( 'NONE', #51666, .T. ) ;
#45990=DIRECTION ( 'NONE',  ( 0.000000000000000000, 1.000000000000000000, 0.000000000000000000 ) ) ;
#45991=EDGE_LOOP ( 'NONE', ( #83080, #55277, #35315, #19362 ) ) ;
#45993=DIRECTION ( 'NONE',  ( 0.000000000000000000, 1.000000000000000000, 0.000000000000000000 ) ) ;
#45994=DIRECTION ( 'NONE',  ( -0.000000000000000000, 1.000000000000000000, -0.000000000000000000 ) ) ;
#45995=LINE ( 'NONE', #8607, #106354 ) ;
#45996=CARTESIAN_POINT ( 'NONE',  ( -0.4500000000000402012, 2.500000000000000000, 2.165063509461097713 ) ) ;
#45997=CARTESIAN_POINT ( 'NONE',  ( -9.150000000000011013, 2.500000000000000000, -5.702370205355745014 ) ) ;
#45998=EDGE_LOOP ( 'NONE', ( #126808, #68203, #65812, #116993 ) ) ;
#45999=ORIENTED_EDGE ( 'NONE', *, *, #78998, .F. ) ;
#46000=FACE_OUTER_BOUND ( 'NONE', #26756, .T. ) ;
#46001=AXIS2_PLACEMENT_3D ( 'NONE', #119659, #50289, #39844 ) ;
#46002=ORIENTED_EDGE ( 'NONE', *, *, #16879, .F. ) ;
#46003=DIRECTION ( 'NONE',  ( -0.000000000000000000, 1.000000000000000000, -0.000000000000000000 ) ) ;
#46004=DIRECTION ( 'NONE',  ( 0.000000000000000000, 0.000000000000000000, 1.000000000000000000 ) ) ;
#46005=EDGE_CURVE ( 'NONE', #69398, #99498, #41993, .T. ) ;
#46006=VECTOR ( 'NONE', #103786, 1000.000000000000000 ) ;
#46007=CONICAL_SURFACE ( 'NONE', #112899, 0.1000000000000000472, 0.003490658503988666988 ) ;
#46008=ORIENTED_EDGE ( 'NONE', *, *, #24588, .F. ) ;
#46010=CARTESIAN_POINT ( 'NONE',  ( 3.349999999999944578, 12.50000000000000000, -5.802370205355749988 ) ) ;
#46011=PLANE ( 'NONE',  #125976 ) ;
#46013=CARTESIAN_POINT ( 'NONE',  ( 4.999999999999936939, 2.500000000000000000, -3.537306695894649966 ) ) ;
#46014=VERTEX_POINT ( 'NONE', #43294 ) ;
#46015=CONICAL_SURFACE ( 'NONE', #81517, 0.1000000000000000472, 0.003490658503988666988 ) ;
#46016=CIRCLE ( 'NONE', #31352, 0.06509327318403745899 ) ;
#46017=DIRECTION ( 'NONE',  ( 0.000000000000000000, -0.000000000000000000, 1.000000000000000000 ) ) ;
#46018=DIRECTION ( 'NONE',  ( -4.274815082592931898E-19, -0.9999939076577903929, -0.003490651415223739937 ) ) ;
#46019=VERTEX_POINT ( 'NONE', #102208 ) ;
#46020=ADVANCED_FACE ( 'NONE', ( #122491 ), #74888, .T. ) ;
#46021=EDGE_CURVE ( 'NONE', #1757, #23452, #18444, .T. ) ;
#46022=EDGE_CURVE ( 'NONE', #103763, #15166, #102076, .T. ) ;
#46023=CARTESIAN_POINT ( 'NONE',  ( -13.09999999999999076, 12.50000000000000000, 3.983716857408420964 ) ) ;
#46024=EDGE_CURVE ( 'NONE', #83715, #24243, #37242, .T. ) ;
#46025=CARTESIAN_POINT ( 'NONE',  ( 13.94999999999989448, 12.50000000000000000, -2.446380397790840266 ) ) ;
#46026=DIRECTION ( 'NONE',  ( 0.000000000000000000, 0.000000000000000000, 1.000000000000000000 ) ) ;
#46027=ORIENTED_EDGE ( 'NONE', *, *, #67216, .T. ) ;
#46028=CARTESIAN_POINT ( 'NONE',  ( -6.900000000000019007, 2.500000000000000000, -4.576537180435978236 ) ) ;
#46029=EDGE_LOOP ( 'NONE', ( #25154, #42149 ) ) ;
#46030=CARTESIAN_POINT ( 'NONE',  ( -12.09999999999999609, 12.50000000000000000, 0.06509327318403916596 ) ) ;
#46031=CARTESIAN_POINT ( 'NONE',  ( 3.099999999999945022, 2.500000000000000000, -0.3464101615137783474 ) ) ;
#46032=ADVANCED_FACE ( 'NONE', ( #34109 ), #5898, .T. ) ;
#46033=DIRECTION ( 'NONE',  ( -4.274815082592931898E-19, -0.9999939076577903929, -0.003490651415223739937 ) ) ;
#46034=ORIENTED_EDGE ( 'NONE', *, *, #102303, .F. ) ;
#46035=ADVANCED_FACE ( 'NONE', ( #53738 ), #94296, .T. ) ;
#46036=AXIS2_PLACEMENT_3D ( 'NONE', #37892, #128224, #116443 ) ;
#46037=DIRECTION ( 'NONE',  ( -0.000000000000000000, 1.000000000000000000, -0.000000000000000000 ) ) ;
#46038=EDGE_CURVE ( 'NONE', #86983, #128651, #58175, .T. ) ;
#46039=AXIS2_PLACEMENT_3D ( 'NONE', #22148, #49025, #20838 ) ;
#46040=DIRECTION ( 'NONE',  ( 0.000000000000000000, 1.000000000000000000, 0.000000000000000000 ) ) ;
#46041=ORIENTED_EDGE ( 'NONE', *, *, #48543, .T. ) ;
#46042=EDGE_LOOP ( 'NONE', ( #109773, #103620, #20371, #49815 ) ) ;
#46043=VECTOR ( 'NONE', #2518, 1000.000000000000000 ) ;
#46044=DIRECTION ( 'NONE',  ( -4.274815082592931898E-19, -0.9999939076577903929, -0.003490651415223739937 ) ) ;
#46045=ORIENTED_EDGE ( 'NONE', *, *, #20566, .F. ) ;
#46046=CARTESIAN_POINT ( 'NONE',  ( 9.799999999999915445, 2.500000000000000000, -4.676537180435977881 ) ) ;
#46047=CARTESIAN_POINT ( 'NONE',  ( -4.600000000000028066, 12.50000000000000000, -5.088040615133791356 ) ) ;
#46048=VERTEX_POINT ( 'NONE', #84317 ) ;
#46049=CIRCLE ( 'NONE', #96198, 0.06509327318403745899 ) ;
#46050=FACE_OUTER_BOUND ( 'NONE', #122334, .T. ) ;
#46051=DIRECTION ( 'NONE',  ( 0.000000000000000000, -0.9999939076577903929, 0.003490651415223739937 ) ) ;
#46052=ORIENTED_EDGE ( 'NONE', *, *, #121368, .F. ) ;
#46053=AXIS2_PLACEMENT_3D ( 'NONE', #117130, #107332, #57602 ) ;
#46054=CARTESIAN_POINT ( 'NONE',  ( 10.59999999999990905, 2.500000000000000000, -3.983716857408426293 ) ) ;
#46055=DIRECTION ( 'NONE',  ( -0.000000000000000000, 1.000000000000000000, -0.000000000000000000 ) ) ;
#46056=CIRCLE ( 'NONE', #75368, 0.09999999999999999167 ) ;
#46057=CARTESIAN_POINT ( 'NONE',  ( 9.799999999999918998, 2.500000000000000000, -0.3464101615137782364 ) ) ;
#46058=CARTESIAN_POINT ( 'NONE',  ( -6.250000000000015987, 12.50000000000000000, 5.802370205355744659 ) ) ;
#46059=DIRECTION ( 'NONE',  ( 0.000000000000000000, 0.000000000000000000, -1.000000000000000000 ) ) ;
#46060=AXIS2_PLACEMENT_3D ( 'NONE', #121039, #81748, #101409 ) ;
#46061=ORIENTED_EDGE ( 'NONE', *, *, #7238, .T. ) ;
#46062=VERTEX_POINT ( 'NONE', #102034 ) ;
#46063=EDGE_LOOP ( 'NONE', ( #72511, #1164 ) ) ;
#46064=EDGE_LOOP ( 'NONE', ( #27109, #105137, #70777, #53699 ) ) ;
#46065=DIRECTION ( 'NONE',  ( -0.000000000000000000, 1.000000000000000000, -0.000000000000000000 ) ) ;
#46066=DIRECTION ( 'NONE',  ( 0.000000000000000000, 1.000000000000000000, 0.000000000000000000 ) ) ;
#46067=DIRECTION ( 'NONE',  ( 0.000000000000000000, -0.000000000000000000, 1.000000000000000000 ) ) ;
#46068=EDGE_LOOP ( 'NONE', ( #111445, #77169, #72666, #20823 ) ) ;
#46069=FACE_BOUND ( 'NONE', #1443, .T. ) ;
#46070=CARTESIAN_POINT ( 'NONE',  ( 14.59999999999989484, 12.50000000000000000, -2.276824562219559311E-15 ) ) ;
#46071=CARTESIAN_POINT ( 'NONE',  ( 5.449999999999934452, 12.50000000000000000, 2.165063509461097713 ) ) ;
#46072=ADVANCED_FACE ( 'NONE', ( #104596 ), #81152, .T. ) ;
#46073=DIRECTION ( 'NONE',  ( 0.000000000000000000, 0.000000000000000000, -1.000000000000000000 ) ) ;
#46074=CARTESIAN_POINT ( 'NONE',  ( 1.249999999999986899, 12.50000000000000000, 6.495190528383297135 ) ) ;
#46075=ADVANCED_FACE ( 'NONE', ( #45058 ), #33132, .T. ) ;
#46076=CARTESIAN_POINT ( 'NONE',  ( -5.200000000000024158, 2.500000000000000000, -4.776537180435977525 ) ) ;
#46077=DIRECTION ( 'NONE',  ( -0.000000000000000000, 1.000000000000000000, -0.000000000000000000 ) ) ;
#46078=DIRECTION ( 'NONE',  ( 0.000000000000000000, 0.000000000000000000, 1.000000000000000000 ) ) ;
#46079=FACE_OUTER_BOUND ( 'NONE', #21603, .T. ) ;
#46080=DIRECTION ( 'NONE',  ( 0.000000000000000000, -0.9999939076577903929, 0.003490651415223739937 ) ) ;
#46081=CARTESIAN_POINT ( 'NONE',  ( 8.549999999999924327, 2.500000000000000000, 1.918653347947321564 ) ) ;
#46082=EDGE_CURVE ( 'NONE', #24019, #110675, #44392, .T. ) ;
#46083=ORIENTED_EDGE ( 'NONE', *, *, #66259, .F. ) ;
#46084=EDGE_LOOP ( 'NONE', ( #39044, #32386, #50353, #53123 ) ) ;
#46085=VERTEX_POINT ( 'NONE', #93501 ) ;
#46086=ORIENTED_EDGE ( 'NONE', *, *, #94030, .F. ) ;
#46087=FACE_OUTER_BOUND ( 'NONE', #32510, .T. ) ;
#46088=EDGE_LOOP ( 'NONE', ( #789, #11043, #96400, #36824 ) ) ;
#46089=DIRECTION ( 'NONE',  ( 0.000000000000000000, 1.000000000000000000, 0.000000000000000000 ) ) ;
#46090=CIRCLE ( 'NONE', #123431, 0.09999999999999982514 ) ;
#46091=ORIENTED_EDGE ( 'NONE', *, *, #62821, .F. ) ;
#46092=VERTEX_POINT ( 'NONE', #2513 ) ;
#46093=CARTESIAN_POINT ( 'NONE',  ( 3.749999999999978684, 2.500000000000000000, -2.165063509461101710 ) ) ;
#46094=CIRCLE ( 'NONE', #14673, 0.09999999999999982514 ) ;
#46095=DIRECTION ( 'NONE',  ( -0.000000000000000000, -1.000000000000000000, -0.000000000000000000 ) ) ;
#46096=DIRECTION ( 'NONE',  ( 0.000000000000000000, 0.000000000000000000, 1.000000000000000000 ) ) ;
#46097=DIRECTION ( 'NONE',  ( 0.000000000000000000, 0.000000000000000000, -1.000000000000000000 ) ) ;
#46098=PLANE ( 'NONE',  #116615 ) ;
#46099=ORIENTED_EDGE ( 'NONE', *, *, #105752, .F. ) ;
#46100=ORIENTED_EDGE ( 'NONE', *, *, #25069, .F. ) ;
#46101=ORIENTED_EDGE ( 'NONE', *, *, #39824, .T. ) ;
#46102=VERTEX_POINT ( 'NONE', #12349 ) ;
#46103=DIRECTION ( 'NONE',  ( 0.000000000000000000, 1.000000000000000000, 0.000000000000000000 ) ) ;
#46104=ORIENTED_EDGE ( 'NONE', *, *, #50563, .F. ) ;
#46105=ORIENTED_EDGE ( 'NONE', *, *, #102331, .F. ) ;
#46106=CARTESIAN_POINT ( 'NONE',  ( 8.349999999999919709, 2.500000000000000000, -1.372243186433550033 ) ) ;
#46107=DIRECTION ( 'NONE',  ( 0.000000000000000000, -0.000000000000000000, 1.000000000000000000 ) ) ;
#46108=CARTESIAN_POINT ( 'NONE',  ( 5.199999999999935341, 2.500000000000000000, -0.3464101615137783474 ) ) ;
#46109=ADVANCED_FACE ( 'NONE', ( #64673 ), #100113, .T. ) ;
#46110=DIRECTION ( 'NONE',  ( 0.000000000000000000, 1.000000000000000000, 0.000000000000000000 ) ) ;
#46111=CARTESIAN_POINT ( 'NONE',  ( 4.999999999999933387, 2.500000000000000000, 5.122947341949749323 ) ) ;
#46112=DIRECTION ( 'NONE',  ( 0.000000000000000000, 0.000000000000000000, 1.000000000000000000 ) ) ;
#46113=VERTEX_POINT ( 'NONE', #92196 ) ;
#46114=DIRECTION ( 'NONE',  ( 0.000000000000000000, 0.000000000000000000, 1.000000000000000000 ) ) ;
#46115=AXIS2_PLACEMENT_3D ( 'NONE', #58038, #35810, #117557 ) ;
#46117=CARTESIAN_POINT ( 'NONE',  ( 4.349999999999941025, 12.50000000000000000, -6.083687093685488989 ) ) ;
#46118=VERTEX_POINT ( 'NONE', #53583 ) ;
#46119=DIRECTION ( 'NONE',  ( 0.000000000000000000, -0.000000000000000000, 1.000000000000000000 ) ) ;
#46120=DIRECTION ( 'NONE',  ( 0.000000000000000000, -0.9999939076577903929, 0.003490651415223739937 ) ) ;
#46121=ADVANCED_FACE ( 'NONE', ( #52931 ), #116819, .T. ) ;
#46122=ORIENTED_EDGE ( 'NONE', *, *, #84766, .T. ) ;
#46123=DIRECTION ( 'NONE',  ( 0.000000000000000000, -0.000000000000000000, 1.000000000000000000 ) ) ;
#46125=FACE_OUTER_BOUND ( 'NONE', #6734, .T. ) ;
#46126=ORIENTED_EDGE ( 'NONE', *, *, #12910, .F. ) ;
#46127=VECTOR ( 'NONE', #36531, 1000.000000000000000 ) ;
#46128=LINE ( 'NONE', #125966, #23642 ) ;
#46129=EDGE_LOOP ( 'NONE', ( #60495, #16507, #7580, #55358 ) ) ;
#46130=EDGE_CURVE ( 'NONE', #14663, #70719, #49960, .T. ) ;
#46131=VERTEX_POINT ( 'NONE', #43137 ) ;
#46132=CARTESIAN_POINT ( 'NONE',  ( 6.699999999999928235, 2.500000000000000000, 0.09999999999999772959 ) ) ;
#46133=DIRECTION ( 'NONE',  ( -4.274815082592931898E-19, -0.9999939076577903929, -0.003490651415223739937 ) ) ;
#46135=CARTESIAN_POINT ( 'NONE',  ( -12.49999999999995914, 12.50000000000000000, -4.265033745738161741 ) ) ;
#46136=CONICAL_SURFACE ( 'NONE', #12755, 0.1000000000000002554, 0.003490658503988666988 ) ;
#46137=CIRCLE ( 'NONE', #85832, 0.1000000000000000056 ) ;
#46138=DIRECTION ( 'NONE',  ( 0.000000000000000000, 0.000000000000000000, 1.000000000000000000 ) ) ;
#46139=CARTESIAN_POINT ( 'NONE',  ( 9.149999999999916866, 2.500000000000000000, 5.702370205355745014 ) ) ;
#46140=AXIS2_PLACEMENT_3D ( 'NONE', #4453, #15582, #7044 ) ;
#46141=ORIENTED_EDGE ( 'NONE', *, *, #88119, .F. ) ;
#46142=CARTESIAN_POINT ( 'NONE',  ( 65.39885637503600435, 3.129858735933689573, -5.811318689367469759 ) ) ;
#46143=EDGE_CURVE ( 'NONE', #124287, #88819, #3953, .T. ) ;
#46144=ORIENTED_EDGE ( 'NONE', *, *, #20211, .F. ) ;
#46145=CIRCLE ( 'NONE', #62881, 0.1000000000000002554 ) ;
#46146=CARTESIAN_POINT ( 'NONE',  ( -13.94999999999998863, 2.500000000000000000, 2.511473670974877503 ) ) ;
#46147=CARTESIAN_POINT ( 'NONE',  ( -8.550000000000014921, 2.500000000000000000, -6.248780366869521430 ) ) ;
#46148=LINE ( 'NONE', #48743, #14581 ) ;
#46149=EDGE_LOOP ( 'NONE', ( #125086, #113694, #58622, #52333 ) ) ;
#46150=EDGE_CURVE ( 'NONE', #25156, #79978, #23462, .T. ) ;
#46151=CARTESIAN_POINT ( 'NONE',  ( -7.100000000000018296, 12.50000000000000000, -0.06509327318403980434 ) ) ;
#46152=CARTESIAN_POINT ( 'NONE',  ( -6.450000000000017941, 2.500000000000000000, -2.411473670974877859 ) ) ;
#46153=ADVANCED_FACE ( 'NONE', ( #5103 ), #35281, .T. ) ;
#46154=EDGE_CURVE ( 'NONE', #98777, #85834, #112634, .T. ) ;
#46155=EDGE_CURVE ( 'NONE', #82690, #111766, #129384, .T. ) ;
#46156=EDGE_CURVE ( 'NONE', #100484, #123441, #10227, .T. ) ;
#46157=ORIENTED_EDGE ( 'NONE', *, *, #118396, .F. ) ;
#46158=DIRECTION ( 'NONE',  ( 0.000000000000000000, -0.9999939076577903929, 0.003490651415223739937 ) ) ;
#46159=ORIENTED_EDGE ( 'NONE', *, *, #78360, .F. ) ;
#46160=ORIENTED_EDGE ( 'NONE', *, *, #117855, .T. ) ;
#46161=DIRECTION ( 'NONE',  ( -0.000000000000000000, 1.000000000000000000, -0.000000000000000000 ) ) ;
#46162=EDGE_CURVE ( 'NONE', #75844, #104306, #108416, .T. ) ;
#46163=AXIS2_PLACEMENT_3D ( 'NONE', #44836, #35028, #74931 ) ;
#46164=AXIS2_PLACEMENT_3D ( 'NONE', #100511, #61901, #101816 ) ;
#46165=EDGE_CURVE ( 'NONE', #33390, #30210, #85433, .T. ) ;
#46168=DIRECTION ( 'NONE',  ( 0.000000000000000000, -0.000000000000000000, 1.000000000000000000 ) ) ;
#46169=CARTESIAN_POINT ( 'NONE',  ( 12.89999999999990266, 2.500000000000000000, 3.737306695894644371 ) ) ;
#46170=ORIENTED_EDGE ( 'NONE', *, *, #100734, .F. ) ;
#46171=EDGE_CURVE ( 'NONE', #53159, #110767, #14276, .T. ) ;
#46172=CONICAL_SURFACE ( 'NONE', #56616, 0.1000000000000000472, 0.003490658503988666988 ) ;
#46173=FACE_BOUND ( 'NONE', #123867, .T. ) ;
#46174=EDGE_CURVE ( 'NONE', #79117, #110068, #4434, .T. ) ;
#46175=DIRECTION ( 'NONE',  ( 0.000000000000000000, 1.000000000000000000, 0.000000000000000000 ) ) ;
#46176=ORIENTED_EDGE ( 'NONE', *, *, #71286, .T. ) ;
#46177=AXIS2_PLACEMENT_3D ( 'NONE', #31148, #2961, #40972 ) ;
#46178=FACE_OUTER_BOUND ( 'NONE', #81121, .T. ) ;
#46179=EDGE_CURVE ( 'NONE', #68357, #40294, #79193, .T. ) ;
#46180=CARTESIAN_POINT ( 'NONE',  ( 1.899999999999951283, 2.500000000000000000, -0.4464101615137782142 ) ) ;
#46181=EDGE_CURVE ( 'NONE', #76087, #53767, #20596, .T. ) ;
#46182=ORIENTED_EDGE ( 'NONE', *, *, #69473, .T. ) ;
#46183=ORIENTED_EDGE ( 'NONE', *, *, #54314, .F. ) ;
#46184=ORIENTED_EDGE ( 'NONE', *, *, #71291, .F. ) ;
#46185=DIRECTION ( 'NONE',  ( 0.000000000000000000, 0.000000000000000000, 1.000000000000000000 ) ) ;
#46186=FACE_OUTER_BOUND ( 'NONE', #28379, .T. ) ;
#46187=DIRECTION ( 'NONE',  ( 0.000000000000000000, 1.000000000000000000, 0.000000000000000000 ) ) ;
#46188=FACE_BOUND ( 'NONE', #71623, .T. ) ;
#46189=ORIENTED_EDGE ( 'NONE', *, *, #23770, .T. ) ;
#46191=CARTESIAN_POINT ( 'NONE',  ( 1.849999999999949685, 2.500000000000000000, 1.818653347947321475 ) ) ;
#46192=DIRECTION ( 'NONE',  ( 0.000000000000000000, -0.9999939076577903929, 0.003490651415223739937 ) ) ;
#46193=CIRCLE ( 'NONE', #119350, 0.09999999999999999167 ) ;
#46194=DIRECTION ( 'NONE',  ( 0.000000000000000000, 0.000000000000000000, 1.000000000000000000 ) ) ;
#46195=CARTESIAN_POINT ( 'NONE',  ( 9.549999999999915445, 2.500000000000000000, 6.495190528383297135 ) ) ;
#46196=PLANE ( 'NONE',  #125978 ) ;
#46197=DIRECTION ( 'NONE',  ( 0.000000000000000000, 0.000000000000000000, 1.000000000000000000 ) ) ;
#46199=VECTOR ( 'NONE', #128918, 1000.000000000000000 ) ;
#46200=CONICAL_SURFACE ( 'NONE', #6457, 0.1000000000000002554, 0.003490658503988666988 ) ;
#46201=CARTESIAN_POINT ( 'NONE',  ( 2.099999999999950351, 2.500000000000000000, -0.6928203230275541413 ) ) ;
#46202=ORIENTED_EDGE ( 'NONE', *, *, #91688, .T. ) ;
#46203=ORIENTED_EDGE ( 'NONE', *, *, #126053, .F. ) ;
#46205=ORIENTED_EDGE ( 'NONE', *, *, #56764, .T. ) ;
#46206=ORIENTED_EDGE ( 'NONE', *, *, #27799, .T. ) ;
#46207=CARTESIAN_POINT ( 'NONE',  ( -10.85000000000000142, 12.50000000000000000, -2.165063509461097713 ) ) ;
#46208=CARTESIAN_POINT ( 'NONE',  ( -3.350000000000028955, 2.500000000000000000, 5.702370205355745014 ) ) ;
#46209=ORIENTED_EDGE ( 'NONE', *, *, #42125, .T. ) ;
#46210=FACE_BOUND ( 'NONE', #53982, .T. ) ;
#46211=CONICAL_SURFACE ( 'NONE', #58741, 0.09999999999999982514, 0.003490658503988666988 ) ;
#46212=DIRECTION ( 'NONE',  ( 0.000000000000000000, 0.000000000000000000, 1.000000000000000000 ) ) ;
#46213=CIRCLE ( 'NONE', #48274, 0.1000000000000002554 ) ;
#46214=EDGE_CURVE ( 'NONE', #22803, #74283, #91700, .T. ) ;
#46215=DIRECTION ( 'NONE',  ( 0.000000000000000000, 0.000000000000000000, 1.000000000000000000 ) ) ;
#46216=EDGE_CURVE ( 'NONE', #97917, #10224, #93760, .T. ) ;
#46217=FACE_OUTER_BOUND ( 'NONE', #114396, .T. ) ;
#46218=DIRECTION ( 'NONE',  ( 0.000000000000000000, 1.000000000000000000, 0.000000000000000000 ) ) ;
#46219=DIRECTION ( 'NONE',  ( 0.000000000000000000, 0.000000000000000000, 1.000000000000000000 ) ) ;
#46220=EDGE_LOOP ( 'NONE', ( #75777, #71559 ) ) ;
#46221=DIRECTION ( 'NONE',  ( 0.000000000000000000, 0.000000000000000000, -1.000000000000000000 ) ) ;
#46222=CIRCLE ( 'NONE', #62945, 0.06509327318403745899 ) ;
#46223=VERTEX_POINT ( 'NONE', #126825 ) ;
#46224=AXIS2_PLACEMENT_3D ( 'NONE', #20599, #31709, #60546 ) ;
#46225=ORIENTED_EDGE ( 'NONE', *, *, #90938, .T. ) ;
#46226=ORIENTED_EDGE ( 'NONE', *, *, #101290, .T. ) ;
#46227=CARTESIAN_POINT ( 'NONE',  ( -5.650000000000023448, 12.50000000000000000, -1.818653347947326138 ) ) ;
#46228=LINE ( 'NONE', #125437, #24642 ) ;
#46229=CARTESIAN_POINT ( 'NONE',  ( 0.8499999999999553468, 12.50000000000000000, 1.537336459617582918 ) ) ;
#46230=ORIENTED_EDGE ( 'NONE', *, *, #86460, .F. ) ;
#46231=FACE_OUTER_BOUND ( 'NONE', #34633, .T. ) ;
#46232=CIRCLE ( 'NONE', #108908, 0.06509327318403743123 ) ;
#46233=CARTESIAN_POINT ( 'NONE',  ( 13.54999999999989946, 2.500000000000000000, 2.511473670974873507 ) ) ;
#46234=DIRECTION ( 'NONE',  ( 0.000000000000000000, 0.000000000000000000, 1.000000000000000000 ) ) ;
#46235=AXIS2_PLACEMENT_3D ( 'NONE', #101104, #21246, #51383 ) ;
#46236=VECTOR ( 'NONE', #88779, 1000.000000000000000 ) ;
#46238=DIRECTION ( 'NONE',  ( 0.000000000000000000, 0.000000000000000000, 1.000000000000000000 ) ) ;
#46239=LINE ( 'NONE', #86144, #24448 ) ;
#46240=VERTEX_POINT ( 'NONE', #76436 ) ;
#46241=DIRECTION ( 'NONE',  ( -0.000000000000000000, -1.000000000000000000, -0.000000000000000000 ) ) ;
#46242=ORIENTED_EDGE ( 'NONE', *, *, #78037, .T. ) ;
#46243=VERTEX_POINT ( 'NONE', #6366 ) ;
#46244=DIRECTION ( 'NONE',  ( -0.000000000000000000, -1.000000000000000000, -0.000000000000000000 ) ) ;
#46245=FACE_OUTER_BOUND ( 'NONE', #47248, .T. ) ;
#46246=FACE_OUTER_BOUND ( 'NONE', #83193, .T. ) ;
#46247=ORIENTED_EDGE ( 'NONE', *, *, #16989, .F. ) ;
#46248=ORIENTED_EDGE ( 'NONE', *, *, #112200, .F. ) ;
#46249=EDGE_CURVE ( 'NONE', #64623, #41154, #102166, .T. ) ;
#46250=DIRECTION ( 'NONE',  ( 0.000000000000000000, -0.000000000000000000, 1.000000000000000000 ) ) ;
#46251=CARTESIAN_POINT ( 'NONE',  ( 32.26057503264689075, 3.190811010352110344, -3.146285318386026209 ) ) ;
#46252=FACE_OUTER_BOUND ( 'NONE', #11965, .T. ) ;
#46254=VERTEX_POINT ( 'NONE', #47622 ) ;
#46255=VECTOR ( 'NONE', #24087, 1000.000000000000000 ) ;
#46256=CIRCLE ( 'NONE', #69231, 0.06509327318403745899 ) ;
#46257=CARTESIAN_POINT ( 'NONE',  ( 10.84999999999990905, 12.50000000000000000, 1.472243186433545459 ) ) ;
#46258=ORIENTED_EDGE ( 'NONE', *, *, #83082, .F. ) ;
#46259=CARTESIAN_POINT ( 'NONE',  ( 11.24999999999990585, 2.500000000000000000, -5.802370205355749988 ) ) ;
#46260=CIRCLE ( 'NONE', #90155, 0.06509327318403745899 ) ;
#46261=FACE_OUTER_BOUND ( 'NONE', #129426, .T. ) ;
#46262=VERTEX_POINT ( 'NONE', #125525 ) ;
#46263=DIRECTION ( 'NONE',  ( 0.000000000000000000, 0.000000000000000000, 1.000000000000000000 ) ) ;
#46264=CONICAL_SURFACE ( 'NONE', #90157, 0.1000000000000002554, 0.003490658503988666988 ) ;
#46265=CARTESIAN_POINT ( 'NONE',  ( -5.200000000000020606, 2.500000000000000000, 4.083716857408421497 ) ) ;
#46266=DIRECTION ( 'NONE',  ( 0.000000000000000000, 0.000000000000000000, 1.000000000000000000 ) ) ;
#46267=AXIS2_PLACEMENT_3D ( 'NONE', #15329, #36302, #66382 ) ;
#46268=EDGE_CURVE ( 'NONE', #107707, #9138, #22765, .T. ) ;
#46269=ADVANCED_FACE ( 'NONE', ( #15565 ), #110473, .T. ) ;
#46270=LINE ( 'NONE', #127420, #102295 ) ;
#46271=ORIENTED_EDGE ( 'NONE', *, *, #95989, .T. ) ;
#46272=DIRECTION ( 'NONE',  ( -0.000000000000000000, 1.000000000000000000, -0.000000000000000000 ) ) ;
#46273=CARTESIAN_POINT ( 'NONE',  ( 0.6499999999999566125, 2.500000000000000000, -6.841600689897077814 ) ) ;
#46274=EDGE_LOOP ( 'NONE', ( #62452, #72455, #61629, #83609 ) ) ;
#46275=ORIENTED_EDGE ( 'NONE', *, *, #50726, .T. ) ;
#46276=ADVANCED_FACE ( 'NONE', ( #106529 ), #127218, .T. ) ;
#46278=CARTESIAN_POINT ( 'NONE',  ( -6.250000000000021316, 2.500000000000000000, -1.472243186433550122 ) ) ;
#46279=CARTESIAN_POINT ( 'NONE',  ( 2.499999999999983569, 2.500000000000000000, -0.1000000000000022815 ) ) ;
#46280=DIRECTION ( 'NONE',  ( -0.000000000000000000, -1.000000000000000000, -0.000000000000000000 ) ) ;
#46281=CARTESIAN_POINT ( 'NONE',  ( -6.650000000000018119, 2.500000000000000000, -2.957883832488653830 ) ) ;
#46282=CARTESIAN_POINT ( 'NONE',  ( -1.650000000000035216, 12.50000000000000000, -5.802370205355749988 ) ) ;
#46283=DIRECTION ( 'NONE',  ( -0.000000000000000000, 1.000000000000000000, -0.000000000000000000 ) ) ;
#46284=DIRECTION ( 'NONE',  ( 0.000000000000000000, 0.000000000000000000, 1.000000000000000000 ) ) ;
#46285=CARTESIAN_POINT ( 'NONE',  ( -10.80000000000000249, 12.50000000000000000, -4.330127018922197202 ) ) ;
#46286=DIRECTION ( 'NONE',  ( -4.274815082592931898E-19, -0.9999939076577903929, -0.003490651415223739937 ) ) ;
#46287=AXIS2_PLACEMENT_3D ( 'NONE', #124228, #105225, #94759 ) ;
#46288=VERTEX_POINT ( 'NONE', #37796 ) ;
#46289=CIRCLE ( 'NONE', #50497, 0.06509327318403745899 ) ;
#46290=ORIENTED_EDGE ( 'NONE', *, *, #39421, .F. ) ;
#46291=DIRECTION ( 'NONE',  ( -0.000000000000000000, 1.000000000000000000, -0.000000000000000000 ) ) ;
#46292=ORIENTED_EDGE ( 'NONE', *, *, #88725, .T. ) ;
#46293=FACE_OUTER_BOUND ( 'NONE', #53429, .T. ) ;
#46294=CARTESIAN_POINT ( 'NONE',  ( 1.449999999999951772, 12.50000000000000000, -6.148780366869526226 ) ) ;
#46295=DIRECTION ( 'NONE',  ( 0.000000000000000000, 0.000000000000000000, -1.000000000000000000 ) ) ;
#46296=AXIS2_PLACEMENT_3D ( 'NONE', #35344, #126298, #115150 ) ;
#46297=ORIENTED_EDGE ( 'NONE', *, *, #50622, .T. ) ;
#46298=CARTESIAN_POINT ( 'NONE',  ( 18.70618316910015011, -2.558637580971261816, -2.503050677946357272 ) ) ;
#46299=ADVANCED_FACE ( 'NONE', ( #87528 ), #31079, .T. ) ;
#46300=CONICAL_SURFACE ( 'NONE', #50811, 0.1000000000000000472, 0.003490658503988666988 ) ;
#46301=DIRECTION ( 'NONE',  ( 0.000000000000000000, 0.000000000000000000, -1.000000000000000000 ) ) ;
#46302=LINE ( 'NONE', #7010, #100352 ) ;
#46303=VERTEX_POINT ( 'NONE', #86230 ) ;
#46304=EDGE_CURVE ( 'NONE', #56986, #32850, #14315, .T. ) ;
#46305=EDGE_CURVE ( 'NONE', #73985, #22876, #7023, .T. ) ;
#46306=DIRECTION ( 'NONE',  ( -0.000000000000000000, -1.000000000000000000, -0.000000000000000000 ) ) ;
#46307=AXIS2_PLACEMENT_3D ( 'NONE', #86736, #87371, #78875 ) ;
#46308=ORIENTED_EDGE ( 'NONE', *, *, #3190, .T. ) ;
#46309=VECTOR ( 'NONE', #86750, 1000.000000000000000 ) ;
#46310=ORIENTED_EDGE ( 'NONE', *, *, #492, .F. ) ;
#46311=ORIENTED_EDGE ( 'NONE', *, *, #24902, .T. ) ;
#46312=ORIENTED_EDGE ( 'NONE', *, *, #29726, .F. ) ;
#46313=LINE ( 'NONE', #65299, #69608 ) ;
#46314=EDGE_CURVE ( 'NONE', #6359, #21428, #56762, .T. ) ;
#46315=EDGE_CURVE ( 'NONE', #125682, #93509, #37169, .T. ) ;
#46316=EDGE_CURVE ( 'NONE', #125373, #21022, #24802, .T. ) ;
#46317=CIRCLE ( 'NONE', #106950, 0.06509327318403745899 ) ;
#46318=LINE ( 'NONE', #39113, #38158 ) ;
#46319=DIRECTION ( 'NONE',  ( 0.000000000000000000, 0.000000000000000000, -1.000000000000000000 ) ) ;
#46320=CARTESIAN_POINT ( 'NONE',  ( -6.450000000000019718, 12.50000000000000000, -6.148780366869526226 ) ) ;
#46321=EDGE_LOOP ( 'NONE', ( #47683, #59283, #16409, #10780 ) ) ;
#46322=ADVANCED_FACE ( 'NONE', ( #115700 ), #18535, .T. ) ;
#46323=CIRCLE ( 'NONE', #67136, 0.1000000000000002554 ) ;
#46324=CIRCLE ( 'NONE', #125725, 0.06509327318403741736 ) ;
#46325=DIRECTION ( 'NONE',  ( 0.000000000000000000, 0.000000000000000000, 1.000000000000000000 ) ) ;
#46327=FACE_OUTER_BOUND ( 'NONE', #99075, .T. ) ;
#46328=CARTESIAN_POINT ( 'NONE',  ( 16.56576425165006228, -2.499999999999998668, -6.084390597445814564 ) ) ;
#46329=DIRECTION ( 'NONE',  ( -0.000000000000000000, -1.000000000000000000, -0.000000000000000000 ) ) ;
#46330=CARTESIAN_POINT ( 'NONE',  ( 18.09676523922663449, -2.526776815559105938, 2.684906793687434234 ) ) ;
#46331=EDGE_CURVE ( 'NONE', #74045, #110749, #74972, .T. ) ;
#46332=EDGE_LOOP ( 'NONE', ( #73673, #58081 ) ) ;
#46333=ORIENTED_EDGE ( 'NONE', *, *, #12475, .F. ) ;
#46334=ORIENTED_EDGE ( 'NONE', *, *, #13941, .F. ) ;
#46335=DIRECTION ( 'NONE',  ( 0.000000000000000000, 0.000000000000000000, -1.000000000000000000 ) ) ;
#46336=DIRECTION ( 'NONE',  ( -4.274815082592931898E-19, -0.9999939076577903929, -0.003490651415223739937 ) ) ;
#46337=DIRECTION ( 'NONE',  ( 0.000000000000000000, 0.000000000000000000, 1.000000000000000000 ) ) ;
#46338=FACE_BOUND ( 'NONE', #27060, .T. ) ;
#46339=DIRECTION ( 'NONE',  ( -0.000000000000000000, -1.000000000000000000, -0.000000000000000000 ) ) ;
#46340=DIRECTION ( 'NONE',  ( -0.000000000000000000, -1.000000000000000000, -0.000000000000000000 ) ) ;
#46341=DIRECTION ( 'NONE',  ( 0.000000000000000000, -0.000000000000000000, 1.000000000000000000 ) ) ;
#46342=CIRCLE ( 'NONE', #6603, 0.06509327318403745899 ) ;
#46343=AXIS2_PLACEMENT_3D ( 'NONE', #8929, #58695, #109732 ) ;
#46345=AXIS2_PLACEMENT_3D ( 'NONE', #50003, #212, #40167 ) ;
#46346=FACE_OUTER_BOUND ( 'NONE', #52003, .T. ) ;
#46347=DIRECTION ( 'NONE',  ( 0.000000000000000000, 1.000000000000000000, 0.000000000000000000 ) ) ;
#46348=FACE_OUTER_BOUND ( 'NONE', #108727, .T. ) ;
#46350=VERTEX_POINT ( 'NONE', #27976 ) ;
#46351=EDGE_LOOP ( 'NONE', ( #76782, #94096 ) ) ;
#46352=ORIENTED_EDGE ( 'NONE', *, *, #96176, .T. ) ;
#46353=CONICAL_SURFACE ( 'NONE', #15030, 0.09999999999999982514, 0.003490658503988666988 ) ;
#46354=CONICAL_SURFACE ( 'NONE', #23363, 0.1000000000000002554, 0.003490658503988666988 ) ;
#46355=DIRECTION ( 'NONE',  ( 0.000000000000000000, 0.000000000000000000, -1.000000000000000000 ) ) ;
#46356=FACE_BOUND ( 'NONE', #51831, .T. ) ;
#46358=AXIS2_PLACEMENT_3D ( 'NONE', #77588, #117494, #38342 ) ;
#46359=CARTESIAN_POINT ( 'NONE',  ( -9.400000000000009237, 12.50000000000000000, -4.676537180435974328 ) ) ;
#46360=ADVANCED_FACE ( 'NONE', ( #25380 ), #95998, .T. ) ;
#46361=ORIENTED_EDGE ( 'NONE', *, *, #27799, .F. ) ;
#46362=CARTESIAN_POINT ( 'NONE',  ( -5.850000000000018296, 2.500000000000000000, 2.757883832488649656 ) ) ;
#46363=DIRECTION ( 'NONE',  ( -0.000000000000000000, -1.000000000000000000, -0.000000000000000000 ) ) ;
#46364=ORIENTED_EDGE ( 'NONE', *, *, #6548, .T. ) ;
#46365=DIRECTION ( 'NONE',  ( 0.000000000000000000, 1.000000000000000000, 0.000000000000000000 ) ) ;
#46366=DIRECTION ( 'NONE',  ( -0.000000000000000000, -1.000000000000000000, -0.000000000000000000 ) ) ;
#46367=ADVANCED_FACE ( 'NONE', ( #120230 ), #22859, .T. ) ;
#46368=VERTEX_POINT ( 'NONE', #41687 ) ;
#46369=DIRECTION ( 'NONE',  ( -0.000000000000000000, 1.000000000000000000, -0.000000000000000000 ) ) ;
#46370=CARTESIAN_POINT ( 'NONE',  ( -9.999999999999971578, 2.500000000000000000, -4.430127018922197735 ) ) ;
#46371=CIRCLE ( 'NONE', #6636, 0.06509327318403745899 ) ;
#46372=AXIS2_PLACEMENT_3D ( 'NONE', #109389, #20375, #18436 ) ;
#46373=VERTEX_POINT ( 'NONE', #58730 ) ;
#46374=CARTESIAN_POINT ( 'NONE',  ( -9.600000000000006750, 2.500000000000000000, 5.122947341949749323 ) ) ;
#46375=FACE_OUTER_BOUND ( 'NONE', #73775, .T. ) ;
#46376=ORIENTED_EDGE ( 'NONE', *, *, #8312, .F. ) ;
#46377=CARTESIAN_POINT ( 'NONE',  ( -1.250000000000036193, 2.500000000000000000, 1.472243186433545459 ) ) ;
#46378=ORIENTED_EDGE ( 'NONE', *, *, #81961, .T. ) ;
#46379=VERTEX_POINT ( 'NONE', #80953 ) ;
#46380=DIRECTION ( 'NONE',  ( 0.000000000000000000, 0.000000000000000000, -1.000000000000000000 ) ) ;
#46381=CIRCLE ( 'NONE', #6646, 0.09999999999999982514 ) ;
#46382=VERTEX_POINT ( 'NONE', #50210 ) ;
#46383=CARTESIAN_POINT ( 'NONE',  ( -2.300000000000033573, 2.500000000000000000, -3.883716857408426648 ) ) ;
#46384=CIRCLE ( 'NONE', #111308, 0.1000000000000000472 ) ;
#46385=CARTESIAN_POINT ( 'NONE',  ( -10.65000000000000391, 12.50000000000000000, -1.818653347947322141 ) ) ;
#46386=AXIS2_PLACEMENT_3D ( 'NONE', #43421, #123251, #72229 ) ;
#46387=ORIENTED_EDGE ( 'NONE', *, *, #12606, .T. ) ;
#46388=VECTOR ( 'NONE', #112956, 1000.000000000000000 ) ;
#46389=CARTESIAN_POINT ( 'NONE',  ( -5.400000000000024336, 2.500000000000000000, -3.737306695894649700 ) ) ;
#46390=DIRECTION ( 'NONE',  ( 0.000000000000000000, 1.000000000000000000, 0.000000000000000000 ) ) ;
#46391=FACE_OUTER_BOUND ( 'NONE', #58532, .T. ) ;
#46392=PLANE ( 'NONE',  #46597 ) ;
#46393=DIRECTION ( 'NONE',  ( -0.000000000000000000, 1.000000000000000000, -0.000000000000000000 ) ) ;
#46395=VECTOR ( 'NONE', #26534, 1000.000000000000000 ) ;
#46396=VERTEX_POINT ( 'NONE', #101230 ) ;
#46397=AXIS2_PLACEMENT_3D ( 'NONE', #113478, #124602, #23822 ) ;
#46398=EDGE_CURVE ( 'NONE', #99722, #84166, #83492, .T. ) ;
#46399=ORIENTED_EDGE ( 'NONE', *, *, #86939, .F. ) ;
#46400=DIRECTION ( 'NONE',  ( 0.000000000000000000, 0.000000000000000000, 1.000000000000000000 ) ) ;
#46401=CARTESIAN_POINT ( 'NONE',  ( -11.64999999999999680, 12.50000000000000000, 6.495190528383297135 ) ) ;
#46402=CONICAL_SURFACE ( 'NONE', #12946, 0.1000000000000000472, 0.003490658503988666988 ) ;
#46403=AXIS2_PLACEMENT_3D ( 'NONE', #115298, #75393, #94391 ) ;
#46404=LINE ( 'NONE', #54939, #43862 ) ;
#46405=ORIENTED_EDGE ( 'NONE', *, *, #117260, .F. ) ;
#46406=ORIENTED_EDGE ( 'NONE', *, *, #111123, .T. ) ;
#46407=ORIENTED_EDGE ( 'NONE', *, *, #28119, .F. ) ;
#46408=CARTESIAN_POINT ( 'NONE',  ( 5.199999999999935341, 12.50000000000000000, -3.918623584224389056 ) ) ;
#46409=CIRCLE ( 'NONE', #115444, 0.06509327318403745899 ) ;
#46410=CARTESIAN_POINT ( 'NONE',  ( -1.650000000000034772, 2.500000000000000000, 1.372243186433545370 ) ) ;
#46411=EDGE_CURVE ( 'NONE', #37483, #91091, #93845, .T. ) ;
#46412=DIRECTION ( 'NONE',  ( -4.274815082592931898E-19, -0.9999939076577903929, -0.003490651415223739937 ) ) ;
#46414=FACE_OUTER_BOUND ( 'NONE', #93450, .T. ) ;
#46415=AXIS2_PLACEMENT_3D ( 'NONE', #24322, #55707, #15776 ) ;
#46416=DIRECTION ( 'NONE',  ( 0.000000000000000000, -0.000000000000000000, 1.000000000000000000 ) ) ;
#46417=FACE_OUTER_BOUND ( 'NONE', #14872, .T. ) ;
#46418=DIRECTION ( 'NONE',  ( 0.000000000000000000, 0.000000000000000000, -1.000000000000000000 ) ) ;
#46419=CARTESIAN_POINT ( 'NONE',  ( -12.89999999999999147, 12.50000000000000000, 3.637306695894644726 ) ) ;
#46420=EDGE_CURVE ( 'NONE', #80777, #117628, #27041, .T. ) ;
#46421=EDGE_CURVE ( 'NONE', #100844, #88410, #58047, .T. ) ;
#46422=CARTESIAN_POINT ( 'NONE',  ( -5.850000000000022737, 12.50000000000000000, -6.495190528383302464 ) ) ;
#46424=EDGE_CURVE ( 'NONE', #79959, #68225, #79289, .T. ) ;
#46425=FACE_OUTER_BOUND ( 'NONE', #37982, .T. ) ;
#46426=VERTEX_POINT ( 'NONE', #428 ) ;
#46427=VERTEX_POINT ( 'NONE', #10885 ) ;
#46428=EDGE_CURVE ( 'NONE', #7354, #79666, #9623, .T. ) ;
#46429=DIRECTION ( 'NONE',  ( -0.000000000000000000, 1.000000000000000000, -0.000000000000000000 ) ) ;
#46430=CARTESIAN_POINT ( 'NONE',  ( 2.049999999999950084, 12.50000000000000000, -2.165063509461101710 ) ) ;
#46431=DIRECTION ( 'NONE',  ( 0.000000000000000000, 1.000000000000000000, 0.000000000000000000 ) ) ;
#46432=CARTESIAN_POINT ( 'NONE',  ( 6.649999999999928413, 12.50000000000000000, 1.472243186433545459 ) ) ;
#46433=CARTESIAN_POINT ( 'NONE',  ( -4.800000000000022915, 2.500000000000000000, -0.3464101615137783474 ) ) ;
#46434=CARTESIAN_POINT ( 'NONE',  ( -0.2000000000000412836, 2.500000000000000000, 4.576537180435972019 ) ) ;
#46435=CARTESIAN_POINT ( 'NONE',  ( 5.399999999999931966, 12.50000000000000000, 4.330127018922196314 ) ) ;
#46436=EDGE_LOOP ( 'NONE', ( #5426, #49491 ) ) ;
#46437=DIRECTION ( 'NONE',  ( 0.000000000000000000, 0.000000000000000000, -1.000000000000000000 ) ) ;
#46438=AXIS2_PLACEMENT_3D ( 'NONE', #106843, #57771, #28306 ) ;
#46439=CIRCLE ( 'NONE', #35990, 0.1000000000000000472 ) ;
#46440=DIRECTION ( 'NONE',  ( 0.000000000000000000, 0.000000000000000000, -1.000000000000000000 ) ) ;
#46441=ORIENTED_EDGE ( 'NONE', *, *, #66844, .T. ) ;
#46443=VECTOR ( 'NONE', #25516, 1000.000000000000000 ) ;
#46444=CIRCLE ( 'NONE', #117525, 0.06509327318403745899 ) ;
#46445=ORIENTED_EDGE ( 'NONE', *, *, #31848, .F. ) ;
#46446=AXIS2_PLACEMENT_3D ( 'NONE', #14668, #46089, #85983 ) ;
#46447=AXIS2_PLACEMENT_3D ( 'NONE', #36624, #35961, #16293 ) ;
#46448=ORIENTED_EDGE ( 'NONE', *, *, #82356, .T. ) ;
#46449=LINE ( 'NONE', #87023, #4406 ) ;
#46450=DIRECTION ( 'NONE',  ( -0.000000000000000000, -1.000000000000000000, -0.000000000000000000 ) ) ;
#46451=AXIS2_PLACEMENT_3D ( 'NONE', #56099, #96657, #25344 ) ;
#46452=ORIENTED_EDGE ( 'NONE', *, *, #32292, .T. ) ;
#46454=CARTESIAN_POINT ( 'NONE',  ( -1.650000000000034772, 2.500000000000000000, 5.702370205355745014 ) ) ;
#46455=CARTESIAN_POINT ( 'NONE',  ( 2.299999999999947864, 2.500000000000000000, 4.083716857408421497 ) ) ;
#46456=VERTEX_POINT ( 'NONE', #31215 ) ;
#46457=DIRECTION ( 'NONE',  ( -0.000000000000000000, 1.000000000000000000, -0.000000000000000000 ) ) ;
#46458=EDGE_CURVE ( 'NONE', #9494, #79598, #43787, .T. ) ;
#46459=DIRECTION ( 'NONE',  ( 0.000000000000000000, 0.000000000000000000, -1.000000000000000000 ) ) ;
#46460=VERTEX_POINT ( 'NONE', #99944 ) ;
#46461=ORIENTED_EDGE ( 'NONE', *, *, #124796, .F. ) ;
#46462=VERTEX_POINT ( 'NONE', #61312 ) ;
#46463=EDGE_CURVE ( 'NONE', #53157, #81003, #91404, .T. ) ;
#46464=CARTESIAN_POINT ( 'NONE',  ( 2.099999999999950351, 2.500000000000000000, -5.022947341949754119 ) ) ;
#46465=ADVANCED_FACE ( 'NONE', ( #20737 ), #39756, .T. ) ;
#46467=EDGE_CURVE ( 'NONE', #89242, #81079, #20785, .T. ) ;
#46468=CIRCLE ( 'NONE', #119626, 0.09999999999999999167 ) ;
#46469=DIRECTION ( 'NONE',  ( 0.000000000000000000, 1.000000000000000000, 0.000000000000000000 ) ) ;
#46470=EDGE_CURVE ( 'NONE', #122261, #29766, #48921, .T. ) ;
#46471=EDGE_LOOP ( 'NONE', ( #100029, #26189 ) ) ;
#46472=FACE_OUTER_BOUND ( 'NONE', #83037, .T. ) ;
#46474=DIRECTION ( 'NONE',  ( -0.000000000000000000, 1.000000000000000000, -0.000000000000000000 ) ) ;
#46475=CARTESIAN_POINT ( 'NONE',  ( -11.05000000000000249, 2.500000000000000000, -1.918653347947322230 ) ) ;
#46476=CONICAL_SURFACE ( 'NONE', #54889, 0.1000000000000002554, 0.003490658503988666988 ) ;
#46477=EDGE_CURVE ( 'NONE', #57283, #101787, #118977, .T. ) ;
#46478=CIRCLE ( 'NONE', #6747, 0.09999999999999982514 ) ;
#46479=EDGE_LOOP ( 'NONE', ( #97751, #46184 ) ) ;
#46480=EDGE_CURVE ( 'NONE', #119348, #93899, #91792, .T. ) ;
#46481=CARTESIAN_POINT ( 'NONE',  ( -5.850000000000021849, 12.50000000000000000, -7.122917578226816815 ) ) ;
#46482=CIRCLE ( 'NONE', #71620, 0.1000000000000002554 ) ;
#46483=EDGE_LOOP ( 'NONE', ( #25652, #88328 ) ) ;
#46484=ORIENTED_EDGE ( 'NONE', *, *, #51003, .T. ) ;
#46485=ORIENTED_EDGE ( 'NONE', *, *, #45020, .F. ) ;
#46486=DIRECTION ( 'NONE',  ( 0.000000000000000000, 0.000000000000000000, 1.000000000000000000 ) ) ;
#46487=FACE_BOUND ( 'NONE', #93901, .T. ) ;
#46488=DIRECTION ( 'NONE',  ( 0.000000000000000000, 0.000000000000000000, 1.000000000000000000 ) ) ;
#46489=DIRECTION ( 'NONE',  ( 0.000000000000000000, 0.000000000000000000, 1.000000000000000000 ) ) ;
#46491=CIRCLE ( 'NONE', #119653, 0.06509327318403745899 ) ;
#46492=CARTESIAN_POINT ( 'NONE',  ( 1.249999999999988454, 2.500000000000000000, -2.065063509461102065 ) ) ;
#46493=AXIS2_PLACEMENT_3D ( 'NONE', #55736, #105492, #96292 ) ;
#46494=ORIENTED_EDGE ( 'NONE', *, *, #104388, .T. ) ;
#46495=CARTESIAN_POINT ( 'NONE',  ( -4.350000000000027178, 2.500000000000000000, -6.248780366869526759 ) ) ;
#46497=PLANE ( 'NONE',  #103005 ) ;
#46498=AXIS2_PLACEMENT_3D ( 'NONE', #32707, #2550, #32058 ) ;
#46499=CARTESIAN_POINT ( 'NONE',  ( -13.09999999999999076, 2.500000000000000000, 3.883716857408421319 ) ) ;
#46500=VERTEX_POINT ( 'NONE', #29277 ) ;
#46501=DIRECTION ( 'NONE',  ( 0.000000000000000000, 0.000000000000000000, 1.000000000000000000 ) ) ;
#46502=CARTESIAN_POINT ( 'NONE',  ( 5.449999999999936229, 12.50000000000000000, 6.495190528383297135 ) ) ;
#46503=AXIS2_PLACEMENT_3D ( 'NONE', #71318, #32075, #11106 ) ;
#46504=EDGE_LOOP ( 'NONE', ( #112644, #72924, #98525, #104476 ) ) ;
#46505=FACE_OUTER_BOUND ( 'NONE', #40271, .T. ) ;
#46506=DIRECTION ( 'NONE',  ( 0.000000000000000000, 0.000000000000000000, 1.000000000000000000 ) ) ;
#46507=FACE_BOUND ( 'NONE', #122716, .T. ) ;
#46508=DIRECTION ( 'NONE',  ( -0.000000000000000000, -1.000000000000000000, -0.000000000000000000 ) ) ;
#46509=ORIENTED_EDGE ( 'NONE', *, *, #73045, .F. ) ;
#46510=DIRECTION ( 'NONE',  ( 0.000000000000000000, 0.000000000000000000, 1.000000000000000000 ) ) ;
#46511=CARTESIAN_POINT ( 'NONE',  ( -15.19999999999998330, 2.500000000000000000, 0.3464101615137758494 ) ) ;
#46512=ORIENTED_EDGE ( 'NONE', *, *, #62405, .T. ) ;
#46513=ORIENTED_EDGE ( 'NONE', *, *, #41790, .T. ) ;
#46514=CONICAL_SURFACE ( 'NONE', #53081, 0.09999999999999999167, 0.003490658503988666988 ) ;
#46516=ORIENTED_EDGE ( 'NONE', *, *, #46162, .F. ) ;
#46518=DIRECTION ( 'NONE',  ( 0.000000000000000000, 0.000000000000000000, 1.000000000000000000 ) ) ;
#46519=EDGE_CURVE ( 'NONE', #83167, #98725, #58361, .T. ) ;
#46520=AXIS2_PLACEMENT_3D ( 'NONE', #19969, #70351, #100455 ) ;
#46521=CARTESIAN_POINT ( 'NONE',  ( -3.749999999999994671, 12.50000000000000000, -6.430097255199264339 ) ) ;
#46522=AXIS2_PLACEMENT_3D ( 'NONE', #72013, #111929, #43205 ) ;
#46523=AXIS2_PLACEMENT_3D ( 'NONE', #73641, #92652, #71723 ) ;
#46524=FACE_OUTER_BOUND ( 'NONE', #44098, .T. ) ;
#46525=CONICAL_SURFACE ( 'NONE', #119694, 0.1000000000000000472, 0.003490658503988666988 ) ;
#46526=EDGE_LOOP ( 'NONE', ( #127718, #14052 ) ) ;
#46528=LINE ( 'NONE', #126395, #98793 ) ;
#46529=DIRECTION ( 'NONE',  ( -0.000000000000000000, -1.000000000000000000, -0.000000000000000000 ) ) ;
#46530=FACE_OUTER_BOUND ( 'NONE', #2244, .T. ) ;
#46531=AXIS2_PLACEMENT_3D ( 'NONE', #27389, #107257, #122566 ) ;
#46532=DIRECTION ( 'NONE',  ( 0.000000000000000000, 0.000000000000000000, -1.000000000000000000 ) ) ;
#46533=AXIS2_PLACEMENT_3D ( 'NONE', #50705, #70348, #19964 ) ;
#46534=VERTEX_POINT ( 'NONE', #71773 ) ;
#46535=CARTESIAN_POINT ( 'NONE',  ( 0.8499999999999545697, 12.50000000000000000, -1.472243186433550122 ) ) ;
#46536=ORIENTED_EDGE ( 'NONE', *, *, #47795, .F. ) ;
#46537=CARTESIAN_POINT ( 'NONE',  ( 6.649999999999931966, 2.500000000000000000, -7.288010851410854585 ) ) ;
#46538=DIRECTION ( 'NONE',  ( 0.000000000000000000, 0.000000000000000000, -1.000000000000000000 ) ) ;
#46539=AXIS2_PLACEMENT_3D ( 'NONE', #42951, #90727, #61928 ) ;
#46540=ORIENTED_EDGE ( 'NONE', *, *, #12480, .T. ) ;
#46541=FACE_OUTER_BOUND ( 'NONE', #41533, .T. ) ;
#46542=CARTESIAN_POINT ( 'NONE',  ( 17.50000000000000000, -2.500000000000000000, -3.999999999999998224 ) ) ;
#46544=CARTESIAN_POINT ( 'NONE',  ( -14.14999999999998614, 2.500000000000000000, -2.265063509461099578 ) ) ;
#46545=EDGE_LOOP ( 'NONE', ( #44973, #33600, #85088, #8825 ) ) ;
#46546=LINE ( 'NONE', #66191, #108021 ) ;
#46547=DIRECTION ( 'NONE',  ( 0.000000000000000000, -0.9999939076577903929, 0.003490651415223739937 ) ) ;
#46550=CARTESIAN_POINT ( 'NONE',  ( 1.849999999999948130, 2.500000000000000000, 6.248780366869520542 ) ) ;
#46551=AXIS2_PLACEMENT_3D ( 'NONE', #72274, #34288, #102371 ) ;
#46552=ORIENTED_EDGE ( 'NONE', *, *, #3488, .T. ) ;
#46553=EDGE_LOOP ( 'NONE', ( #73077, #88107, #10134, #42803 ) ) ;
#46554=DIRECTION ( 'NONE',  ( 0.000000000000000000, 1.000000000000000000, 0.000000000000000000 ) ) ;
#46555=ORIENTED_EDGE ( 'NONE', *, *, #21176, .T. ) ;
#46556=FACE_OUTER_BOUND ( 'NONE', #56251, .T. ) ;
#46557=EDGE_LOOP ( 'NONE', ( #50802, #105717 ) ) ;
#46558=VERTEX_POINT ( 'NONE', #73061 ) ;
#46559=VERTEX_POINT ( 'NONE', #14118 ) ;
#46560=DIRECTION ( 'NONE',  ( 0.000000000000000000, 1.000000000000000000, 0.000000000000000000 ) ) ;
#46561=AXIS2_PLACEMENT_3D ( 'NONE', #83974, #72256, #31671 ) ;
#46563=DIRECTION ( 'NONE',  ( 0.000000000000000000, 0.000000000000000000, 1.000000000000000000 ) ) ;
#46564=ADVANCED_FACE ( 'NONE', ( #14746 ), #14409, .T. ) ;
#46565=AXIS2_PLACEMENT_3D ( 'NONE', #64244, #104173, #74071 ) ;
#46566=CARTESIAN_POINT ( 'NONE',  ( -9.800000000000006040, 12.50000000000000000, 0.3464101615137735735 ) ) ;
#46568=DIRECTION ( 'NONE',  ( -0.000000000000000000, -1.000000000000000000, -0.000000000000000000 ) ) ;
#46569=CARTESIAN_POINT ( 'NONE',  ( -11.25000000000000178, 12.50000000000000000, -1.472243186433546125 ) ) ;
#46570=CARTESIAN_POINT ( 'NONE',  ( -10.84999999999999964, 12.50000000000000000, 7.188010851410848723 ) ) ;
#46571=EDGE_CURVE ( 'NONE', #118622, #50743, #45829, .T. ) ;
#46572=ORIENTED_EDGE ( 'NONE', *, *, #81631, .F. ) ;
#46573=CIRCLE ( 'NONE', #4791, 0.06509327318403745899 ) ;
#46574=EDGE_CURVE ( 'NONE', #23743, #46243, #18627, .T. ) ;
#46575=CIRCLE ( 'NONE', #84224, 0.09999999999999982514 ) ;
#46576=CARTESIAN_POINT ( 'NONE',  ( 1.449999999999952660, 2.500000000000000000, -6.941600689897078347 ) ) ;
#46577=ORIENTED_EDGE ( 'NONE', *, *, #46420, .F. ) ;
#46579=ORIENTED_EDGE ( 'NONE', *, *, #43207, .T. ) ;
#46580=ORIENTED_EDGE ( 'NONE', *, *, #39097, .F. ) ;
#46581=ORIENTED_EDGE ( 'NONE', *, *, #35533, .T. ) ;
#46582=EDGE_CURVE ( 'NONE', #58440, #15244, #110567, .T. ) ;
#46583=DIRECTION ( 'NONE',  ( -0.000000000000000000, 1.000000000000000000, -0.000000000000000000 ) ) ;
#46584=EDGE_CURVE ( 'NONE', #54447, #37927, #22041, .T. ) ;
#46585=EDGE_CURVE ( 'NONE', #29513, #17807, #1898, .T. ) ;
#46586=VERTEX_POINT ( 'NONE', #61957 ) ;
#46587=ORIENTED_EDGE ( 'NONE', *, *, #48374, .F. ) ;
#46589=AXIS2_PLACEMENT_3D ( 'NONE', #90271, #68712, #614 ) ;
#46590=AXIS2_PLACEMENT_3D ( 'NONE', #48458, #57642, #17019 ) ;
#46591=DIRECTION ( 'NONE',  ( -0.000000000000000000, -1.000000000000000000, -0.000000000000000000 ) ) ;
#46592=DIRECTION ( 'NONE',  ( -0.000000000000000000, -1.000000000000000000, -0.000000000000000000 ) ) ;
#46593=DIRECTION ( 'NONE',  ( 0.000000000000000000, 0.000000000000000000, 1.000000000000000000 ) ) ;
#46594=CONICAL_SURFACE ( 'NONE', #67502, 0.09999999999999982514, 0.003490658503988666988 ) ;
#46595=DIRECTION ( 'NONE',  ( 0.000000000000000000, 1.000000000000000000, 0.000000000000000000 ) ) ;
#46596=AXIS2_PLACEMENT_3D ( 'NONE', #16307, #57553, #58212 ) ;
#46597=AXIS2_PLACEMENT_3D ( 'NONE', #34678, #93579, #15637 ) ;
#46598=DIRECTION ( 'NONE',  ( 0.000000000000000000, 1.000000000000000000, 0.000000000000000000 ) ) ;
#46599=EDGE_LOOP ( 'NONE', ( #52206, #31345 ) ) ;
#46600=EDGE_CURVE ( 'NONE', #26024, #9406, #10315, .T. ) ;
#46601=CIRCLE ( 'NONE', #23617, 0.06509327318403745899 ) ;
#46602=DIRECTION ( 'NONE',  ( 0.000000000000000000, 0.000000000000000000, -1.000000000000000000 ) ) ;
#46603=VERTEX_POINT ( 'NONE', #42315 ) ;
#46604=CARTESIAN_POINT ( 'NONE',  ( 3.949999999999941558, 12.50000000000000000, -6.148780366869526226 ) ) ;
#46605=VERTEX_POINT ( 'NONE', #104446 ) ;
#46606=CIRCLE ( 'NONE', #119765, 0.1000000000000002554 ) ;
#46607=CARTESIAN_POINT ( 'NONE',  ( -12.29999999999999716, 2.500000000000000000, 0.3464101615137776813 ) ) ;
#46608=ORIENTED_EDGE ( 'NONE', *, *, #52310, .F. ) ;
#46609=EDGE_LOOP ( 'NONE', ( #75438, #42350 ) ) ;
#46610=CARTESIAN_POINT ( 'NONE',  ( 1.249999999999952038, 12.50000000000000000, -1.472243186433550122 ) ) ;
#46611=CARTESIAN_POINT ( 'NONE',  ( -9.800000000000004263, 2.500000000000000000, -0.3464101615137783474 ) ) ;
#46612=DIRECTION ( 'NONE',  ( 0.000000000000000000, 0.000000000000000000, 1.000000000000000000 ) ) ;
#46613=FACE_OUTER_BOUND ( 'NONE', #91122, .T. ) ;
#46614=CARTESIAN_POINT ( 'NONE',  ( -13.29999999999999005, 2.500000000000000000, -0.09999999999999815981 ) ) ;
#46615=EDGE_LOOP ( 'NONE', ( #57648, #12222, #47626, #111983 ) ) ;
#46616=CARTESIAN_POINT ( 'NONE',  ( -9.800000000000004263, 12.50000000000000000, 4.048810130592458201 ) ) ;
#46617=FACE_OUTER_BOUND ( 'NONE', #60770, .T. ) ;
#46618=VECTOR ( 'NONE', #43873, 1000.000000000000000 ) ;
#46619=EDGE_CURVE ( 'NONE', #117732, #113146, #68807, .T. ) ;
#46620=CARTESIAN_POINT ( 'NONE',  ( 1.449999999999951328, 12.50000000000000000, 2.511473670974873507 ) ) ;
#46621=CARTESIAN_POINT ( 'NONE',  ( -7.900000000000014566, 12.50000000000000000, -0.6928203230275541413 ) ) ;
#46622=CARTESIAN_POINT ( 'NONE',  ( -8.550000000000011369, 2.500000000000000000, 1.818653347947321475 ) ) ;
#46624=AXIS2_PLACEMENT_3D ( 'NONE', #35864, #6363, #14893 ) ;
#46625=CONICAL_SURFACE ( 'NONE', #57086, 0.09999999999999999167, 0.003490658503988666988 ) ;
#46626=ORIENTED_EDGE ( 'NONE', *, *, #108512, .T. ) ;
#46627=VECTOR ( 'NONE', #115786, 1000.000000000000000 ) ;
#46628=AXIS2_PLACEMENT_3D ( 'NONE', #2988, #42938, #82852 ) ;
#46629=ADVANCED_FACE ( 'NONE', ( #52136 ), #112729, .T. ) ;
#46630=DIRECTION ( 'NONE',  ( 0.000000000000000000, 1.000000000000000000, 0.000000000000000000 ) ) ;
#46631=ADVANCED_FACE ( 'NONE', ( #4939 ), #52091, .T. ) ;
#46632=EDGE_CURVE ( 'NONE', #96281, #93919, #129476, .T. ) ;
#46633=ORIENTED_EDGE ( 'NONE', *, *, #56536, .F. ) ;
#46634=DIRECTION ( 'NONE',  ( 0.000000000000000000, 0.000000000000000000, 1.000000000000000000 ) ) ;
#46635=DIRECTION ( 'NONE',  ( 0.000000000000000000, 0.000000000000000000, 1.000000000000000000 ) ) ;
#46636=CIRCLE ( 'NONE', #103070, 0.06509327318403745899 ) ;
#46637=AXIS2_PLACEMENT_3D ( 'NONE', #42969, #10863, #102501 ) ;
#46638=EDGE_CURVE ( 'NONE', #26852, #60457, #73012, .T. ) ;
#46639=AXIS2_PLACEMENT_3D ( 'NONE', #21909, #111557, #71635 ) ;
#46640=CIRCLE ( 'NONE', #2713, 0.1000000000000000472 ) ;
#46641=EDGE_CURVE ( 'NONE', #108185, #40494, #121035, .T. ) ;
#46642=EDGE_LOOP ( 'NONE', ( #105667, #35233, #49343, #45143 ) ) ;
#46644=LINE ( 'NONE', #108135, #89265 ) ;
#46645=DIRECTION ( 'NONE',  ( -0.000000000000000000, 1.000000000000000000, -0.000000000000000000 ) ) ;
#46646=EDGE_CURVE ( 'NONE', #103825, #106452, #33769, .T. ) ;
#46648=PLANE ( 'NONE',  #7817 ) ;
#46649=ORIENTED_EDGE ( 'NONE', *, *, #22353, .T. ) ;
#46650=CIRCLE ( 'NONE', #55055, 0.09999999999999982514 ) ;
#46651=EDGE_CURVE ( 'NONE', #5985, #30750, #113626, .T. ) ;
#46652=ADVANCED_FACE ( 'NONE', ( #84152 ), #16548, .T. ) ;
#46653=EDGE_CURVE ( 'NONE', #59036, #101170, #89735, .T. ) ;
#46654=CARTESIAN_POINT ( 'NONE',  ( 6.649999999999930189, 2.500000000000000000, -1.372243186433550033 ) ) ;
#46655=DIRECTION ( 'NONE',  ( 0.000000000000000000, 0.000000000000000000, 1.000000000000000000 ) ) ;
#46656=ORIENTED_EDGE ( 'NONE', *, *, #16748, .T. ) ;
#46657=DIRECTION ( 'NONE',  ( 0.000000000000000000, 0.000000000000000000, 1.000000000000000000 ) ) ;
#46658=LINE ( 'NONE', #35559, #85255 ) ;
#46659=ADVANCED_FACE ( 'NONE', ( #96537 ), #127395, .T. ) ;
#46660=CARTESIAN_POINT ( 'NONE',  ( -9.600000000000006750, 2.500000000000000000, -0.7928203230275543412 ) ) ;
#46661=CIRCLE ( 'NONE', #75897, 0.1000000000000000472 ) ;
#46662=ORIENTED_EDGE ( 'NONE', *, *, #119077, .F. ) ;
#46663=DIRECTION ( 'NONE',  ( 0.000000000000000000, -0.000000000000000000, 1.000000000000000000 ) ) ;
#46664=EDGE_LOOP ( 'NONE', ( #76529, #41282, #72574, #9484 ) ) ;
#46665=DIRECTION ( 'NONE',  ( 0.000000000000000000, 1.000000000000000000, 0.000000000000000000 ) ) ;
#46666=FACE_OUTER_BOUND ( 'NONE', #112896, .T. ) ;
#46667=CARTESIAN_POINT ( 'NONE',  ( -0.2000000000000347888, 2.500000000000000000, 0.2464101615137758439 ) ) ;
#46668=AXIS2_PLACEMENT_3D ( 'NONE', #23460, #103966, #35235 ) ;
#46669=VERTEX_POINT ( 'NONE', #117450 ) ;
#46670=CIRCLE ( 'NONE', #126074, 0.06509327318403745899 ) ;
#46671=AXIS2_PLACEMENT_3D ( 'NONE', #62615, #112350, #82897 ) ;
#46672=DIRECTION ( 'NONE',  ( 0.000000000000000000, 0.000000000000000000, 1.000000000000000000 ) ) ;
#46673=DIRECTION ( 'NONE',  ( -1.000000000000000000, -0.000000000000000000, -0.000000000000000000 ) ) ;
#46674=ORIENTED_EDGE ( 'NONE', *, *, #100243, .T. ) ;
#46675=AXIS2_PLACEMENT_3D ( 'NONE', #84348, #7055, #5761 ) ;
#46676=EDGE_LOOP ( 'NONE', ( #19262, #84734, #43082, #96530 ) ) ;
#46678=AXIS2_PLACEMENT_3D ( 'NONE', #52351, #65220, #42558 ) ;
#46679=AXIS2_PLACEMENT_3D ( 'NONE', #45203, #85108, #25530 ) ;
#46680=VERTEX_POINT ( 'NONE', #17993 ) ;
#46681=CARTESIAN_POINT ( 'NONE',  ( -1.650000000000035216, 12.50000000000000000, -5.737276932171712751 ) ) ;
#46682=CARTESIAN_POINT ( 'NONE',  ( -4.350000000000023626, 2.500000000000000000, 2.511473670974873507 ) ) ;
#46683=ORIENTED_EDGE ( 'NONE', *, *, #105746, .T. ) ;
#46684=VERTEX_POINT ( 'NONE', #124732 ) ;
#46685=CARTESIAN_POINT ( 'NONE',  ( -11.64999999999999680, 2.500000000000000000, -2.857883832488649745 ) ) ;
#46686=FACE_OUTER_BOUND ( 'NONE', #89966, .T. ) ;
#46687=VERTEX_POINT ( 'NONE', #7525 ) ;
#46688=CARTESIAN_POINT ( 'NONE',  ( 1.849999999999948130, 12.50000000000000000, 6.148780366869520009 ) ) ;
#46689=CARTESIAN_POINT ( 'NONE',  ( 12.89999999999989910, 2.500000000000000000, -0.7928203230275543412 ) ) ;
#46690=EDGE_CURVE ( 'NONE', #126577, #40083, #119074, .T. ) ;
#46691=AXIS2_PLACEMENT_3D ( 'NONE', #110884, #2215, #42161 ) ;
#46692=CONICAL_SURFACE ( 'NONE', #40451, 0.1000000000000002554, 0.003490658503988666988 ) ;
#46693=AXIS2_PLACEMENT_3D ( 'NONE', #112427, #31299, #111777 ) ;
#46694=DIRECTION ( 'NONE',  ( 0.000000000000000000, 1.000000000000000000, 0.000000000000000000 ) ) ;
#46695=CARTESIAN_POINT ( 'NONE',  ( 4.199999999999939782, 2.500000000000000000, -2.276824562219559311E-15 ) ) ;
#46696=CARTESIAN_POINT ( 'NONE',  ( 3.749999999999942268, 12.50000000000000000, -1.472243186433550122 ) ) ;
#46697=CONICAL_SURFACE ( 'NONE', #719, 0.1000000000000002554, 0.003490658503988666988 ) ;
#46698=DIRECTION ( 'NONE',  ( 0.000000000000000000, 0.000000000000000000, 1.000000000000000000 ) ) ;
#46699=EDGE_LOOP ( 'NONE', ( #57494, #103452, #59559, #28065 ) ) ;
#46700=VERTEX_POINT ( 'NONE', #84802 ) ;
#46701=ORIENTED_EDGE ( 'NONE', *, *, #111327, .T. ) ;
#46702=ORIENTED_EDGE ( 'NONE', *, *, #88816, .F. ) ;
#46703=DIRECTION ( 'NONE',  ( 0.000000000000000000, 0.000000000000000000, 1.000000000000000000 ) ) ;
#46704=CARTESIAN_POINT ( 'NONE',  ( 9.549999999999915445, 12.50000000000000000, 6.560283801567334372 ) ) ;
#46705=LINE ( 'NONE', #25123, #32234 ) ;
#46706=ORIENTED_EDGE ( 'NONE', *, *, #16164, .F. ) ;
#46707=EDGE_CURVE ( 'NONE', #57903, #89650, #68886, .T. ) ;
#46708=FACE_BOUND ( 'NONE', #110475, .T. ) ;
#46709=CARTESIAN_POINT ( 'NONE',  ( -2.100000000000034284, 2.500000000000000000, -2.385244779468109755E-15 ) ) ;
#46710=CARTESIAN_POINT ( 'NONE',  ( -3.750000000000031086, 2.500000000000000000, -5.702370205355749455 ) ) ;
#46711=DIRECTION ( 'NONE',  ( -0.000000000000000000, 1.000000000000000000, -0.000000000000000000 ) ) ;
#46712=DIRECTION ( 'NONE',  ( 0.000000000000000000, 0.000000000000000000, 1.000000000000000000 ) ) ;
#46713=CARTESIAN_POINT ( 'NONE',  ( 8.099999999999921485, 12.50000000000000000, -0.4115034346978157509 ) ) ;
#46714=DIRECTION ( 'NONE',  ( 0.000000000000000000, 1.000000000000000000, 0.000000000000000000 ) ) ;
#46715=DIRECTION ( 'NONE',  ( 0.000000000000000000, 0.000000000000000000, 1.000000000000000000 ) ) ;
#46716=CARTESIAN_POINT ( 'NONE',  ( -13.74999999999995381, 2.500000000000000000, 2.165063509461101265 ) ) ;
#46717=VECTOR ( 'NONE', #35969, 1000.000000000000000 ) ;
#46718=AXIS2_PLACEMENT_3D ( 'NONE', #117529, #58009, #97912 ) ;
#46719=FACE_OUTER_BOUND ( 'NONE', #77117, .T. ) ;
#46720=DIRECTION ( 'NONE',  ( 0.000000000000000000, -0.9999939076577903929, 0.003490651415223739937 ) ) ;
#46721=CONICAL_SURFACE ( 'NONE', #103148, 0.1000000000000002554, 0.003490658503988666988 ) ;
#46722=AXIS2_PLACEMENT_3D ( 'NONE', #65924, #57408, #37131 ) ;
#46723=ORIENTED_EDGE ( 'NONE', *, *, #42782, .T. ) ;
#46724=ORIENTED_EDGE ( 'NONE', *, *, #121331, .T. ) ;
#46725=EDGE_LOOP ( 'NONE', ( #77332, #78268 ) ) ;
#46726=VECTOR ( 'NONE', #97403, 1000.000000000000000 ) ;
#46727=ORIENTED_EDGE ( 'NONE', *, *, #39935, .T. ) ;
#46728=CARTESIAN_POINT ( 'NONE',  ( 12.49999999999993960, 12.50000000000000000, -4.330127018922201643 ) ) ;
#46729=AXIS2_PLACEMENT_3D ( 'NONE', #117540, #28554, #19353 ) ;
#46730=AXIS2_PLACEMENT_3D ( 'NONE', #21173, #62412, #102953 ) ;
#46731=DIRECTION ( 'NONE',  ( 0.000000000000000000, 0.000000000000000000, -1.000000000000000000 ) ) ;
#46732=VERTEX_POINT ( 'NONE', #44897 ) ;
#46733=EDGE_LOOP ( 'NONE', ( #72684, #85228 ) ) ;
#46734=EDGE_LOOP ( 'NONE', ( #105521, #105360, #121781, #23573 ) ) ;
#46735=CARTESIAN_POINT ( 'NONE',  ( -1.700000000000034817, 2.500000000000000000, -4.430127018922202176 ) ) ;
#46736=CONICAL_SURFACE ( 'NONE', #36288, 0.09999999999999982514, 0.003490658503988666988 ) ;
#46737=VECTOR ( 'NONE', #71104, 1000.000000000000000 ) ;
#46738=ADVANCED_FACE ( 'NONE', ( #46830 ), #93945, .T. ) ;
#46739=CARTESIAN_POINT ( 'NONE',  ( 10.30524027349368765, -1.500000000000191402, 9.130939513664339202 ) ) ;
#46740=LINE ( 'NONE', #107591, #104387 ) ;
#46741=PLANE ( 'NONE',  #88629 ) ;
#46742=CONICAL_SURFACE ( 'NONE', #63463, 0.1000000000000002554, 0.003490658503988666988 ) ;
#46743=CARTESIAN_POINT ( 'NONE',  ( -11.84999999999999787, 2.500000000000000000, -6.941600689897074794 ) ) ;
#46744=CIRCLE ( 'NONE', #2823, 0.09999999999999982514 ) ;
#46745=EDGE_LOOP ( 'NONE', ( #65022, #118301 ) ) ;
#46746=EDGE_CURVE ( 'NONE', #59695, #113633, #121127, .T. ) ;
#46747=VERTEX_POINT ( 'NONE', #116191 ) ;
#46749=VERTEX_POINT ( 'NONE', #6861 ) ;
#46750=ADVANCED_FACE ( 'NONE', ( #56614 ), #74990, .T. ) ;
#46751=DIRECTION ( 'NONE',  ( 0.000000000000000000, 0.000000000000000000, 1.000000000000000000 ) ) ;
#46752=EDGE_CURVE ( 'NONE', #107557, #22212, #65141, .T. ) ;
#46754=ADVANCED_FACE ( 'NONE', ( #105075 ), #98132, .T. ) ;
#46755=VERTEX_POINT ( 'NONE', #95280 ) ;
#46756=EDGE_CURVE ( 'NONE', #72001, #102540, #125336, .T. ) ;
#46757=EDGE_CURVE ( 'NONE', #115958, #78678, #86069, .T. ) ;
#46758=VERTEX_POINT ( 'NONE', #37007 ) ;
#46759=CIRCLE ( 'NONE', #7012, 0.06509327318403745899 ) ;
#46760=FACE_OUTER_BOUND ( 'NONE', #76852, .T. ) ;
#46761=CARTESIAN_POINT ( 'NONE',  ( 6.249999999999928946, 12.50000000000000000, 2.857883832488649301 ) ) ;
#46762=DIRECTION ( 'NONE',  ( 0.000000000000000000, -0.000000000000000000, 1.000000000000000000 ) ) ;
#46763=CARTESIAN_POINT ( 'NONE',  ( 14.19999999999989626, 12.50000000000000000, -2.276824562219559311E-15 ) ) ;
#46764=DIRECTION ( 'NONE',  ( 0.000000000000000000, 0.000000000000000000, 1.000000000000000000 ) ) ;
#46765=EDGE_CURVE ( 'NONE', #34089, #22876, #54234, .T. ) ;
#46766=AXIS2_PLACEMENT_3D ( 'NONE', #77076, #57440, #426 ) ;
#46767=ORIENTED_EDGE ( 'NONE', *, *, #91890, .F. ) ;
#46768=CARTESIAN_POINT ( 'NONE',  ( -12.04999999999999716, 12.50000000000000000, -2.165063509461097713 ) ) ;
#46769=CONICAL_SURFACE ( 'NONE', #119918, 0.1000000000000000472, 0.003490658503988666988 ) ;
#46770=EDGE_CURVE ( 'NONE', #37854, #20339, #14497, .T. ) ;
#46772=ADVANCED_FACE ( 'NONE', ( #75612 ), #27175, .T. ) ;
#46773=ORIENTED_EDGE ( 'NONE', *, *, #102731, .T. ) ;
#46774=CARTESIAN_POINT ( 'NONE',  ( 8.549999999999920774, 12.50000000000000000, 6.213873640053559022 ) ) ;
#46776=CARTESIAN_POINT ( 'NONE',  ( -8.550000000000011369, 2.500000000000000000, -2.611473670974877592 ) ) ;
#46777=CARTESIAN_POINT ( 'NONE',  ( 10.44999999999991047, 2.500000000000000000, 2.265063509461097357 ) ) ;
#46778=ORIENTED_EDGE ( 'NONE', *, *, #3486, .T. ) ;
#46779=CARTESIAN_POINT ( 'NONE',  ( -6.249999999999981348, 2.500000000000000000, 2.265063509461097357 ) ) ;
#46780=CARTESIAN_POINT ( 'NONE',  ( -6.050000000000022027, 2.500000000000000000, -1.718653347947326049 ) ) ;
#46781=CIRCLE ( 'NONE', #53037, 0.06509327318403745899 ) ;
#46782=EDGE_LOOP ( 'NONE', ( #13530, #116164, #6283, #75391 ) ) ;
#46783=AXIS2_PLACEMENT_3D ( 'NONE', #102471, #80903, #63193 ) ;
#46784=B_SPLINE_CURVE_WITH_KNOTS ( 'NONE', 3,
 ( #37604, #8120, #97157, #226 ),
 .UNSPECIFIED., .F., .F.,
 ( 4, 4 ),
 ( 0.001845843513054588186, 0.003313552284081220344 ),
 .UNSPECIFIED. ) ;
#46785=AXIS2_PLACEMENT_3D ( 'NONE', #122721, #93910, #13396 ) ;
#46786=DIRECTION ( 'NONE',  ( 0.000000000000000000, -0.9999939076577903929, 0.003490651415223739937 ) ) ;
#46787=ORIENTED_EDGE ( 'NONE', *, *, #127884, .T. ) ;
#46788=VERTEX_POINT ( 'NONE', #46169 ) ;
#46789=DIRECTION ( 'NONE',  ( 0.000000000000000000, 0.000000000000000000, 1.000000000000000000 ) ) ;
#46790=CARTESIAN_POINT ( 'NONE',  ( 10.59999999999990905, 12.50000000000000000, -3.983716857408426293 ) ) ;
#46792=AXIS2_PLACEMENT_3D ( 'NONE', #26598, #116886, #77613 ) ;
#46793=CARTESIAN_POINT ( 'NONE',  ( -7.500000000000001776, 2.500000000000000000, 10.00000000000000178 ) ) ;
#46794=CARTESIAN_POINT ( 'NONE',  ( -6.250000000000017764, 12.50000000000000000, 7.253104124594885960 ) ) ;
#46795=CIRCLE ( 'NONE', #28004, 0.06509327318403745899 ) ;
#46796=CIRCLE ( 'NONE', #63521, 0.1000000000000002554 ) ;
#46797=CARTESIAN_POINT ( 'NONE',  ( -0.6500000000000394351, 2.500000000000000000, 2.511473670974873507 ) ) ;
#46798=AXIS2_PLACEMENT_3D ( 'NONE', #49307, #48004, #38850 ) ;
#46799=EDGE_LOOP ( 'NONE', ( #95674, #106692, #75345, #4557 ) ) ;
#46800=AXIS2_PLACEMENT_3D ( 'NONE', #82762, #120731, #84670 ) ;
#46801=CARTESIAN_POINT ( 'NONE',  ( 10.84999999999990905, 2.500000000000000000, -7.088010851410853519 ) ) ;
#46802=ORIENTED_EDGE ( 'NONE', *, *, #91933, .T. ) ;
#46803=FACE_OUTER_BOUND ( 'NONE', #78220, .T. ) ;
#46804=CARTESIAN_POINT ( 'NONE',  ( -10.45000000000000462, 12.50000000000000000, -6.430097255199260786 ) ) ;
#46805=DIRECTION ( 'NONE',  ( 0.000000000000000000, 0.000000000000000000, 1.000000000000000000 ) ) ;
#46806=EDGE_CURVE ( 'NONE', #20962, #69086, #73105, .T. ) ;
#46807=DIRECTION ( 'NONE',  ( 0.000000000000000000, 0.000000000000000000, 1.000000000000000000 ) ) ;
#46808=DIRECTION ( 'NONE',  ( -4.274815082592931898E-19, -0.9999939076577903929, -0.003490651415223739937 ) ) ;
#46809=ORIENTED_EDGE ( 'NONE', *, *, #81745, .F. ) ;
#46810=EDGE_CURVE ( 'NONE', #72078, #78871, #114853, .T. ) ;
#46811=EDGE_CURVE ( 'NONE', #98383, #24036, #29209, .T. ) ;
#46812=CARTESIAN_POINT ( 'NONE',  ( -13.09999999999999076, 2.500000000000000000, 4.676537180435972552 ) ) ;
#46813=CARTESIAN_POINT ( 'NONE',  ( -9.600000000000006750, 12.50000000000000000, 0.6928203230275494784 ) ) ;
#46814=AXIS2_PLACEMENT_3D ( 'NONE', #39220, #100047, #119043 ) ;
#46815=CONICAL_SURFACE ( 'NONE', #107445, 0.1000000000000000472, 0.003490658503988666988 ) ;
#46816=ORIENTED_EDGE ( 'NONE', *, *, #60059, .F. ) ;
#46817=EDGE_CURVE ( 'NONE', #70962, #62174, #4126, .T. ) ;
#46818=CARTESIAN_POINT ( 'NONE',  ( 11.64999999999990798, 2.500000000000000000, 5.802370205355744659 ) ) ;
#46819=AXIS2_PLACEMENT_3D ( 'NONE', #31066, #122007, #80800 ) ;
#46820=CONICAL_SURFACE ( 'NONE', #71963, 0.09999999999999982514, 0.003490658503988666988 ) ;
#46821=ORIENTED_EDGE ( 'NONE', *, *, #55666, .F. ) ;
#46822=AXIS2_PLACEMENT_3D ( 'NONE', #40207, #41514, #120052 ) ;
#46823=ORIENTED_EDGE ( 'NONE', *, *, #70911, .F. ) ;
#46824=DIRECTION ( 'NONE',  ( 0.000000000000000000, 0.000000000000000000, -1.000000000000000000 ) ) ;
#46825=AXIS2_PLACEMENT_3D ( 'NONE', #45476, #84729, #24529 ) ;
#46826=VECTOR ( 'NONE', #30865, 1000.000000000000000 ) ;
#46827=VERTEX_POINT ( 'NONE', #48117 ) ;
#46829=LINE ( 'NONE', #8805, #69476 ) ;
#46830=FACE_OUTER_BOUND ( 'NONE', #87791, .T. ) ;
#46831=AXIS2_PLACEMENT_3D ( 'NONE', #64033, #75139, #25376 ) ;
#46832=ORIENTED_EDGE ( 'NONE', *, *, #48377, .F. ) ;
#46833=AXIS2_PLACEMENT_3D ( 'NONE', #64916, #114665, #84571 ) ;
#46834=AXIS2_PLACEMENT_3D ( 'NONE', #87089, #68747, #20299 ) ;
#46835=FACE_BOUND ( 'NONE', #54877, .T. ) ;
#46836=DIRECTION ( 'NONE',  ( -0.000000000000000000, -1.000000000000000000, -0.000000000000000000 ) ) ;
#46837=ORIENTED_EDGE ( 'NONE', *, *, #118716, .T. ) ;
#46838=AXIS2_PLACEMENT_3D ( 'NONE', #35348, #104707, #115154 ) ;
#46839=CARTESIAN_POINT ( 'NONE',  ( 3.349999999999941913, 2.500000000000000000, 5.702370205355745014 ) ) ;
#46840=DIRECTION ( 'NONE',  ( 0.000000000000000000, -0.000000000000000000, 1.000000000000000000 ) ) ;
#46841=ADVANCED_FACE ( 'NONE', ( #72107 ), #87663, .T. ) ;
#46843=ORIENTED_EDGE ( 'NONE', *, *, #43037, .T. ) ;
#46844=ORIENTED_EDGE ( 'NONE', *, *, #102331, .T. ) ;
#46845=DIRECTION ( 'NONE',  ( 0.000000000000000000, 0.000000000000000000, -1.000000000000000000 ) ) ;
#46846=VECTOR ( 'NONE', #69595, 1000.000000000000000 ) ;
#46847=DIRECTION ( 'NONE',  ( 0.000000000000000000, 0.000000000000000000, -1.000000000000000000 ) ) ;
#46848=CARTESIAN_POINT ( 'NONE',  ( 14.14999999999989377, 12.50000000000000000, -1.537336459617587581 ) ) ;
#46849=FACE_BOUND ( 'NONE', #60, .T. ) ;
#46850=ORIENTED_EDGE ( 'NONE', *, *, #40606, .F. ) ;
#46851=DIRECTION ( 'NONE',  ( 0.000000000000000000, 1.000000000000000000, 0.000000000000000000 ) ) ;
#46852=CARTESIAN_POINT ( 'NONE',  ( 12.89999999999989910, 2.500000000000000000, 0.7928203230275495672 ) ) ;
#46853=AXIS2_PLACEMENT_3D ( 'NONE', #98823, #39927, #119755 ) ;
#46854=DIRECTION ( 'NONE',  ( -0.000000000000000000, -1.000000000000000000, -0.000000000000000000 ) ) ;
#46855=EDGE_CURVE ( 'NONE', #111888, #84054, #79371, .T. ) ;
#46856=CARTESIAN_POINT ( 'NONE',  ( 2.949999999999943334, 2.500000000000000000, 6.595190528383296780 ) ) ;
#46857=CARTESIAN_POINT ( 'NONE',  ( 12.09999999999990195, 12.50000000000000000, 0.6928203230275494784 ) ) ;
#46858=DIRECTION ( 'NONE',  ( -0.000000000000000000, -1.000000000000000000, -0.000000000000000000 ) ) ;
#46859=CARTESIAN_POINT ( 'NONE',  ( 2.949999999999943334, 2.500000000000000000, 6.495190528383297135 ) ) ;
#46860=CONICAL_SURFACE ( 'NONE', #23884, 0.09999999999999982514, 0.003490658503988666988 ) ;
#46861=CONICAL_SURFACE ( 'NONE', #25928, 0.09999999999999982514, 0.003490658503988666988 ) ;
#46862=EDGE_LOOP ( 'NONE', ( #48975, #84684, #16415, #105869 ) ) ;
#46863=EDGE_LOOP ( 'NONE', ( #22356, #12541 ) ) ;
#46864=EDGE_LOOP ( 'NONE', ( #6179, #16878, #34352, #106996 ) ) ;
#46865=ORIENTED_EDGE ( 'NONE', *, *, #76473, .T. ) ;
#46866=EDGE_LOOP ( 'NONE', ( #51098, #57322 ) ) ;
#46867=DIRECTION ( 'NONE',  ( 0.000000000000000000, 0.000000000000000000, 1.000000000000000000 ) ) ;
#46868=CARTESIAN_POINT ( 'NONE',  ( 1.849999999999948130, 2.500000000000000000, 6.248780366869520542 ) ) ;
#46869=ORIENTED_EDGE ( 'NONE', *, *, #83299, .T. ) ;
#46870=EDGE_CURVE ( 'NONE', #123660, #56688, #122493, .T. ) ;
#46871=FACE_BOUND ( 'NONE', #10713, .T. ) ;
#46872=AXIS2_PLACEMENT_3D ( 'NONE', #57315, #97233, #109641 ) ;
#46873=DIRECTION ( 'NONE',  ( 0.000000000000000000, 0.000000000000000000, 1.000000000000000000 ) ) ;
#46874=VECTOR ( 'NONE', #6851, 1000.000000000000000 ) ;
#46875=CARTESIAN_POINT ( 'NONE',  ( 1.449999999999952660, 2.500000000000000000, -6.841600689897078702 ) ) ;
#46876=CARTESIAN_POINT ( 'NONE',  ( -7.900000000000011013, 2.500000000000000000, 3.637306695894644726 ) ) ;
#46877=CARTESIAN_POINT ( 'NONE',  ( -3.100000000000028955, 12.50000000000000000, 4.741630453620009789 ) ) ;
#46878=CARTESIAN_POINT ( 'NONE',  ( -11.44999999999999751, 2.500000000000000000, 6.248780366869521430 ) ) ;
#46879=VERTEX_POINT ( 'NONE', #88003 ) ;
#46880=CARTESIAN_POINT ( 'NONE',  ( -1.250000000000001554, 2.500000000000000000, 6.395190528383296602 ) ) ;
#46881=EDGE_LOOP ( 'NONE', ( #60166, #74109 ) ) ;
#46883=ORIENTED_EDGE ( 'NONE', *, *, #22251, .T. ) ;
#46884=EDGE_LOOP ( 'NONE', ( #85706, #77474 ) ) ;
#46885=LINE ( 'NONE', #128695, #94431 ) ;
#46886=DIRECTION ( 'NONE',  ( 0.000000000000000000, 1.000000000000000000, 0.000000000000000000 ) ) ;
#46887=DIRECTION ( 'NONE',  ( 1.000000000000000000, 0.000000000000000000, -0.000000000000000000 ) ) ;
#46888=AXIS2_PLACEMENT_3D ( 'NONE', #19831, #59774, #99682 ) ;
#46889=ORIENTED_EDGE ( 'NONE', *, *, #51023, .T. ) ;
#46890=CARTESIAN_POINT ( 'NONE',  ( 7.306656945292924199, 2.499999999999746425, -9.704971168060907871 ) ) ;
#46891=AXIS2_PLACEMENT_3D ( 'NONE', #113002, #23317, #1109 ) ;
#46892=CARTESIAN_POINT ( 'NONE',  ( -10.20000000000000462, 2.500000000000000000, 4.676537180435972552 ) ) ;
#46893=EDGE_CURVE ( 'NONE', #60832, #45836, #47980, .T. ) ;
#46894=LINE ( 'NONE', #5651, #87086 ) ;
#46896=DIRECTION ( 'NONE',  ( 0.000000000000000000, 0.000000000000000000, 1.000000000000000000 ) ) ;
#46897=DIRECTION ( 'NONE',  ( -4.274815082592931898E-19, -0.9999939076577903929, -0.003490651415223739937 ) ) ;
#46898=CARTESIAN_POINT ( 'NONE',  ( -1.900000000000034550, 2.500000000000000000, 4.676537180435972552 ) ) ;
#46899=VERTEX_POINT ( 'NONE', #769 ) ;
#46900=DIRECTION ( 'NONE',  ( -0.000000000000000000, -1.000000000000000000, -0.000000000000000000 ) ) ;
#46901=ADVANCED_FACE ( 'NONE', ( #127953 ), #92368, .T. ) ;
#46902=ORIENTED_EDGE ( 'NONE', *, *, #32335, .F. ) ;
#46903=AXIS2_PLACEMENT_3D ( 'NONE', #1357, #121772, #10528 ) ;
#46904=EDGE_LOOP ( 'NONE', ( #47834, #86956 ) ) ;
#46905=DIRECTION ( 'NONE',  ( -0.000000000000000000, 1.000000000000000000, -0.000000000000000000 ) ) ;
#46906=CIRCLE ( 'NONE', #65664, 0.06509327318403741736 ) ;
#46907=AXIS2_PLACEMENT_3D ( 'NONE', #13425, #53374, #63836 ) ;
#46908=EDGE_CURVE ( 'NONE', #72759, #14578, #60603, .T. ) ;
#46910=CARTESIAN_POINT ( 'NONE',  ( -4.350000000000027178, 12.50000000000000000, -6.148780366869526226 ) ) ;
#46911=ADVANCED_FACE ( 'NONE', ( #51824 ), #20874, .T. ) ;
#46912=EDGE_CURVE ( 'NONE', #28244, #49584, #121830, .T. ) ;
#46913=EDGE_CURVE ( 'NONE', #92549, #23743, #41995, .T. ) ;
#46914=VERTEX_POINT ( 'NONE', #72746 ) ;
#46915=ORIENTED_EDGE ( 'NONE', *, *, #16446, .T. ) ;
#46916=DIRECTION ( 'NONE',  ( -0.000000000000000000, 1.000000000000000000, -0.000000000000000000 ) ) ;
#46917=AXIS2_PLACEMENT_3D ( 'NONE', #59726, #102675, #63411 ) ;
#46918=CIRCLE ( 'NONE', #49072, 0.1000000000000002554 ) ;
#46919=VECTOR ( 'NONE', #2975, 1000.000000000000000 ) ;
#46920=PLANE ( 'NONE',  #68342 ) ;
#46921=EDGE_CURVE ( 'NONE', #102305, #125960, #68384, .T. ) ;
#46922=FACE_OUTER_BOUND ( 'NONE', #29566, .T. ) ;
#46923=ORIENTED_EDGE ( 'NONE', *, *, #96325, .F. ) ;
#46924=VERTEX_POINT ( 'NONE', #112025 ) ;
#46925=EDGE_CURVE ( 'NONE', #90822, #48868, #94028, .T. ) ;
#46926=CARTESIAN_POINT ( 'NONE',  ( -9.150000000000005684, 12.50000000000000000, 7.188010851410848723 ) ) ;
#46927=EDGE_CURVE ( 'NONE', #4486, #119497, #90422, .T. ) ;
#46928=ORIENTED_EDGE ( 'NONE', *, *, #99508, .F. ) ;
#46929=DIRECTION ( 'NONE',  ( 0.000000000000000000, 0.000000000000000000, 1.000000000000000000 ) ) ;
#46930=AXIS2_PLACEMENT_3D ( 'NONE', #109762, #10881, #10268 ) ;
#46931=ADVANCED_FACE ( 'NONE', ( #100893 ), #89817, .T. ) ;
#46932=AXIS2_PLACEMENT_3D ( 'NONE', #12307, #20850, #92158 ) ;
#46933=VECTOR ( 'NONE', #113175, 1000.000000000000000 ) ;
#46934=EDGE_CURVE ( 'NONE', #85762, #13568, #31531, .T. ) ;
#46935=CARTESIAN_POINT ( 'NONE',  ( -7.100000000000013856, 12.50000000000000000, 3.637306695894644726 ) ) ;
#46936=ORIENTED_EDGE ( 'NONE', *, *, #8107, .F. ) ;
#46937=CARTESIAN_POINT ( 'NONE',  ( 5.649999999999932854, 2.500000000000000000, 2.411473670974873862 ) ) ;
#46938=LINE ( 'NONE', #58039, #65095 ) ;
#46939=DIRECTION ( 'NONE',  ( 0.000000000000000000, -0.9999939076577903929, 0.003490651415223739937 ) ) ;
#46940=AXIS2_PLACEMENT_3D ( 'NONE', #45017, #62085, #62728 ) ;
#46941=CARTESIAN_POINT ( 'NONE',  ( 4.549999999999935874, 12.50000000000000000, 6.560283801567334372 ) ) ;
#46942=EDGE_CURVE ( 'NONE', #36299, #6668, #10400, .T. ) ;
#46943=ORIENTED_EDGE ( 'NONE', *, *, #30238, .F. ) ;
#46944=DIRECTION ( 'NONE',  ( -0.000000000000000000, 1.000000000000000000, -0.000000000000000000 ) ) ;
#46945=DIRECTION ( 'NONE',  ( 0.000000000000000000, 1.000000000000000000, 0.000000000000000000 ) ) ;
#46946=ORIENTED_EDGE ( 'NONE', *, *, #26281, .T. ) ;
#46947=EDGE_LOOP ( 'NONE', ( #1032, #106371 ) ) ;
#46949=DIRECTION ( 'NONE',  ( 0.000000000000000000, -0.000000000000000000, 1.000000000000000000 ) ) ;
#46950=FACE_OUTER_BOUND ( 'NONE', #112903, .T. ) ;
#46951=DIRECTION ( 'NONE',  ( 0.000000000000000000, 0.000000000000000000, 1.000000000000000000 ) ) ;
#46952=CONICAL_SURFACE ( 'NONE', #15611, 0.1000000000000002554, 0.003490658503988666988 ) ;
#46953=CARTESIAN_POINT ( 'NONE',  ( -3.150000000000030109, 2.500000000000000000, 1.918653347947321564 ) ) ;
#46954=CARTESIAN_POINT ( 'NONE',  ( 0.8499999999999550138, 2.500000000000000000, -5.702370205355749455 ) ) ;
#46955=LINE ( 'NONE', #38429, #32166 ) ;
#46956=CARTESIAN_POINT ( 'NONE',  ( 5.599999999999931255, 2.500000000000000000, 4.676537180435972552 ) ) ;
#46957=DIRECTION ( 'NONE',  ( 0.000000000000000000, -0.9999939076577903929, 0.003490651415223739937 ) ) ;
#46958=CARTESIAN_POINT ( 'NONE',  ( 13.74999999999989342, 12.50000000000000000, -1.407149913249512663 ) ) ;
#46959=AXIS2_PLACEMENT_3D ( 'NONE', #71295, #43800, #103357 ) ;
#46960=VERTEX_POINT ( 'NONE', #2051 ) ;
#46961=FACE_OUTER_BOUND ( 'NONE', #89112, .T. ) ;
#46962=EDGE_LOOP ( 'NONE', ( #3170, #110384, #118615, #107093 ) ) ;
#46963=DIRECTION ( 'NONE',  ( 0.000000000000000000, 0.000000000000000000, 1.000000000000000000 ) ) ;
#46964=CARTESIAN_POINT ( 'NONE',  ( 11.04999999999990656, 2.500000000000000000, -6.148780366869526226 ) ) ;
#46965=DIRECTION ( 'NONE',  ( 0.000000000000000000, 0.000000000000000000, -1.000000000000000000 ) ) ;
#46966=ORIENTED_EDGE ( 'NONE', *, *, #106100, .T. ) ;
#46967=FACE_OUTER_BOUND ( 'NONE', #78787, .T. ) ;
#46968=AXIS2_PLACEMENT_3D ( 'NONE', #4131, #114107, #112825 ) ;
#46969=EDGE_CURVE ( 'NONE', #96613, #50485, #1989, .T. ) ;
#46970=EDGE_CURVE ( 'NONE', #53584, #128668, #83581, .T. ) ;
#46971=CARTESIAN_POINT ( 'NONE',  ( 4.149999999999938183, 12.50000000000000000, 2.165063509461097713 ) ) ;
#46972=DIRECTION ( 'NONE',  ( 0.000000000000000000, 0.000000000000000000, 1.000000000000000000 ) ) ;
#46973=EDGE_LOOP ( 'NONE', ( #113458, #51579, #109663, #19697 ) ) ;
#46974=LINE ( 'NONE', #45046, #6109 ) ;
#46975=ORIENTED_EDGE ( 'NONE', *, *, #60800, .T. ) ;
#46976=EDGE_CURVE ( 'NONE', #17021, #23771, #58445, .T. ) ;
#46977=CIRCLE ( 'NONE', #34462, 0.1000000000000002554 ) ;
#46978=CONICAL_SURFACE ( 'NONE', #120134, 0.1000000000000000472, 0.003490658503988666988 ) ;
#46979=ORIENTED_EDGE ( 'NONE', *, *, #61871, .F. ) ;
#46980=EDGE_LOOP ( 'NONE', ( #38084, #49850, #72753, #97639 ) ) ;
#46981=ORIENTED_EDGE ( 'NONE', *, *, #45603, .F. ) ;
#46982=DIRECTION ( 'NONE',  ( 0.000000000000000000, 0.000000000000000000, -1.000000000000000000 ) ) ;
#46983=CONICAL_SURFACE ( 'NONE', #44923, 0.1000000000000002554, 0.003490658503988666988 ) ;
#46984=CARTESIAN_POINT ( 'NONE',  ( 9.399999999999915090, 2.500000000000000000, 3.883716857408421319 ) ) ;
#46985=CARTESIAN_POINT ( 'NONE',  ( -6.850000000000013856, 12.50000000000000000, 6.776507416713035248 ) ) ;
#46986=AXIS2_PLACEMENT_3D ( 'NONE', #44249, #104465, #96561 ) ;
#46987=CARTESIAN_POINT ( 'NONE',  ( 11.24999999999991118, 12.50000000000000000, -2.857883832488653741 ) ) ;
#46988=ORIENTED_EDGE ( 'NONE', *, *, #49034, .F. ) ;
#46989=CARTESIAN_POINT ( 'NONE',  ( -7.300000000000013145, 12.50000000000000000, 3.983716857408420076 ) ) ;
#46990=ORIENTED_EDGE ( 'NONE', *, *, #41147, .T. ) ;
#46991=CARTESIAN_POINT ( 'NONE',  ( 23.99354682434742259, -2.839181451644826382, -2.508508607409395186 ) ) ;
#46992=CARTESIAN_POINT ( 'NONE',  ( 15.62920359459681485, -2.499999999999998668, -5.623946225393044784 ) ) ;
#46993=DIRECTION ( 'NONE',  ( 0.000000000000000000, 0.000000000000000000, 1.000000000000000000 ) ) ;
#46994=DIRECTION ( 'NONE',  ( -0.000000000000000000, -1.000000000000000000, -0.000000000000000000 ) ) ;
#46995=ORIENTED_EDGE ( 'NONE', *, *, #124326, .F. ) ;
#46996=VERTEX_POINT ( 'NONE', #53109 ) ;
#46997=ORIENTED_EDGE ( 'NONE', *, *, #46179, .T. ) ;
#46998=AXIS2_PLACEMENT_3D ( 'NONE', #120833, #71735, #43581 ) ;
#46999=ORIENTED_EDGE ( 'NONE', *, *, #121810, .F. ) ;
#47000=LINE ( 'NONE', #126843, #29423 ) ;
#47001=CARTESIAN_POINT ( 'NONE',  ( 48.83367117123161449, 2.320420702480692210, 5.300559035860525903 ) ) ;
#47002=VECTOR ( 'NONE', #80099, 1000.000000000000000 ) ;
#47003=AXIS2_PLACEMENT_3D ( 'NONE', #29197, #8235, #18054 ) ;
#47004=LINE ( 'NONE', #85621, #58673 ) ;
#47005=FACE_BOUND ( 'NONE', #33374, .T. ) ;
#47006=CARTESIAN_POINT ( 'NONE',  ( -10.40000000000000213, 12.50000000000000000, -5.022947341949749678 ) ) ;
#47007=DIRECTION ( 'NONE',  ( 0.000000000000000000, 0.000000000000000000, 1.000000000000000000 ) ) ;
#47008=CARTESIAN_POINT ( 'NONE',  ( -15.19999999999998153, 2.500000000000000000, -0.3464101615137759604 ) ) ;
#47009=FACE_OUTER_BOUND ( 'NONE', #110687, .T. ) ;
#47010=EDGE_CURVE ( 'NONE', #30131, #79994, #2071, .T. ) ;
#47011=CONICAL_SURFACE ( 'NONE', #109788, 0.09999999999999982514, 0.003490658503988666988 ) ;
#47012=CONICAL_SURFACE ( 'NONE', #120160, 0.1000000000000002554, 0.003490658503988666988 ) ;
#47013=AXIS2_PLACEMENT_3D ( 'NONE', #99092, #9418, #49362 ) ;
#47015=CONICAL_SURFACE ( 'NONE', #107646, 0.1000000000000000056, 0.003490658503988666988 ) ;
#47016=DIRECTION ( 'NONE',  ( -0.000000000000000000, 1.000000000000000000, -0.000000000000000000 ) ) ;
#47017=FACE_OUTER_BOUND ( 'NONE', #96591, .T. ) ;
#47018=AXIS2_PLACEMENT_3D ( 'NONE', #118246, #107784, #126787 ) ;
#47019=CIRCLE ( 'NONE', #5231, 0.06509327318403745899 ) ;
#47020=DIRECTION ( 'NONE',  ( 0.000000000000000000, 1.000000000000000000, 0.000000000000000000 ) ) ;
#47021=VERTEX_POINT ( 'NONE', #55676 ) ;
#47022=ORIENTED_EDGE ( 'NONE', *, *, #111159, .T. ) ;
#47023=ORIENTED_EDGE ( 'NONE', *, *, #53286, .T. ) ;
#47024=VERTEX_POINT ( 'NONE', #45870 ) ;
#47025=VECTOR ( 'NONE', #60645, 1000.000000000000000 ) ;
#47026=ADVANCED_FACE ( 'NONE', ( #75951 ), #75246, .T. ) ;
#47027=FACE_OUTER_BOUND ( 'NONE', #80532, .T. ) ;
#47028=EDGE_CURVE ( 'NONE', #97854, #118876, #68986, .T. ) ;
#47029=FACE_BOUND ( 'NONE', #11357, .T. ) ;
#47030=CARTESIAN_POINT ( 'NONE',  ( 8.349999999999923261, 2.500000000000000000, -6.495190528383302464 ) ) ;
#47031=CARTESIAN_POINT ( 'NONE',  ( 0.6499999999999566125, 12.50000000000000000, -6.776507416713039689 ) ) ;
#47032=VERTEX_POINT ( 'NONE', #44572 ) ;
#47033=CARTESIAN_POINT ( 'NONE',  ( -8.750000000000012434, 12.50000000000000000, -5.867463478539781896 ) ) ;
#47035=DIRECTION ( 'NONE',  ( 0.000000000000000000, 0.000000000000000000, 1.000000000000000000 ) ) ;
#47037=VERTEX_POINT ( 'NONE', #115884 ) ;
#47038=DIRECTION ( 'NONE',  ( 0.000000000000000000, -0.9999939076577903929, 0.003490651415223739937 ) ) ;
#47039=CARTESIAN_POINT ( 'NONE',  ( -6.250000000000021316, 12.50000000000000000, -5.737276932171712751 ) ) ;
#47040=ORIENTED_EDGE ( 'NONE', *, *, #119769, .F. ) ;
#47041=DIRECTION ( 'NONE',  ( -0.000000000000000000, -1.000000000000000000, -0.000000000000000000 ) ) ;
#47042=CARTESIAN_POINT ( 'NONE',  ( 5.449999999999936229, 12.50000000000000000, -2.230156782645139391 ) ) ;
#47043=AXIS2_PLACEMENT_3D ( 'NONE', #99978, #18823, #50237 ) ;
#47045=DIRECTION ( 'NONE',  ( 0.000000000000000000, -0.000000000000000000, 1.000000000000000000 ) ) ;
#47046=CARTESIAN_POINT ( 'NONE',  ( 9.399999999999915090, 2.500000000000000000, -4.776537180435977525 ) ) ;
#47047=ORIENTED_EDGE ( 'NONE', *, *, #28012, .F. ) ;
#47048=CARTESIAN_POINT ( 'NONE',  ( -4.200000000000025935, 2.500000000000000000, -0.1000000000000023925 ) ) ;
#47050=EDGE_LOOP ( 'NONE', ( #33017, #48077 ) ) ;
#47051=DIRECTION ( 'NONE',  ( 0.000000000000000000, -0.000000000000000000, 1.000000000000000000 ) ) ;
#47052=VERTEX_POINT ( 'NONE', #14443 ) ;
#47053=CARTESIAN_POINT ( 'NONE',  ( 3.299999999999944755, 12.50000000000000000, -2.385244779468109755E-15 ) ) ;
#47054=FACE_OUTER_BOUND ( 'NONE', #7963, .T. ) ;
#47055=VECTOR ( 'NONE', #53740, 1000.000000000000000 ) ;
#47056=ADVANCED_FACE ( 'NONE', ( #74032 ), #35554, .T. ) ;
#47057=ORIENTED_EDGE ( 'NONE', *, *, #32768, .F. ) ;
#47058=CIRCLE ( 'NONE', #3147, 0.1000000000000002554 ) ;
#47059=CARTESIAN_POINT ( 'NONE',  ( 4.999999999999933387, 12.50000000000000000, 5.022947341949748790 ) ) ;
#47060=VERTEX_POINT ( 'NONE', #115207 ) ;
#47061=DIRECTION ( 'NONE',  ( 0.000000000000000000, 1.000000000000000000, 0.000000000000000000 ) ) ;
#47062=DIRECTION ( 'NONE',  ( 0.000000000000000000, 1.000000000000000000, 0.000000000000000000 ) ) ;
#47063=CARTESIAN_POINT ( 'NONE',  ( -4.600000000000028955, 2.500000000000000000, -4.330127018922201643 ) ) ;
#47064=FACE_OUTER_BOUND ( 'NONE', #118439, .T. ) ;
#47065=ADVANCED_FACE ( 'NONE', ( #83215 ), #118882, .T. ) ;
#47066=CARTESIAN_POINT ( 'NONE',  ( -3.550000000000028244, 12.50000000000000000, 2.446380397790835826 ) ) ;
#47067=EDGE_CURVE ( 'NONE', #87160, #51388, #24287, .T. ) ;
#47068=VERTEX_POINT ( 'NONE', #123135 ) ;
#47069=EDGE_LOOP ( 'NONE', ( #3322, #110334 ) ) ;
#47070=FACE_OUTER_BOUND ( 'NONE', #92097, .T. ) ;
#47071=AXIS2_PLACEMENT_3D ( 'NONE', #99820, #79531, #10144 ) ;
#47072=AXIS2_PLACEMENT_3D ( 'NONE', #74241, #85969, #23861 ) ;
#47073=DIRECTION ( 'NONE',  ( -0.000000000000000000, -1.000000000000000000, -0.000000000000000000 ) ) ;
#47074=EDGE_CURVE ( 'NONE', #76186, #125301, #121209, .T. ) ;
#47075=CARTESIAN_POINT ( 'NONE',  ( 9.199999999999915801, 2.500000000000000000, 4.430127018922196847 ) ) ;
#47076=VERTEX_POINT ( 'NONE', #105430 ) ;
#47077=ORIENTED_EDGE ( 'NONE', *, *, #97458, .T. ) ;
#47078=ADVANCED_FACE ( 'NONE', ( #23636 ), #63574, .T. ) ;
#47079=EDGE_LOOP ( 'NONE', ( #18949, #40235 ) ) ;
#47080=ADVANCED_FACE ( 'NONE', ( #13802 ), #25075, .T. ) ;
#47081=DIRECTION ( 'NONE',  ( 0.000000000000000000, 1.000000000000000000, 0.000000000000000000 ) ) ;
#47082=DIRECTION ( 'NONE',  ( -0.000000000000000000, -1.000000000000000000, -0.000000000000000000 ) ) ;
#47083=FACE_OUTER_BOUND ( 'NONE', #12668, .T. ) ;
#47085=EDGE_CURVE ( 'NONE', #74025, #113934, #112906, .T. ) ;
#47086=DIRECTION ( 'NONE',  ( 0.000000000000000000, 0.000000000000000000, 1.000000000000000000 ) ) ;
#47087=LINE ( 'NONE', #48359, #4236 ) ;
#47089=CARTESIAN_POINT ( 'NONE',  ( 8.349999999999919709, 2.500000000000000000, 7.288010851410849256 ) ) ;
#47090=DIRECTION ( 'NONE',  ( -0.000000000000000000, 1.000000000000000000, -0.000000000000000000 ) ) ;
#47091=VECTOR ( 'NONE', #10509, 1000.000000000000000 ) ;
#47092=CARTESIAN_POINT ( 'NONE',  ( 8.949999999999921130, 12.50000000000000000, -6.906693963081115939 ) ) ;
#47093=EDGE_CURVE ( 'NONE', #122264, #70390, #71049, .T. ) ;
#47094=ORIENTED_EDGE ( 'NONE', *, *, #116899, .F. ) ;
#47095=CONICAL_SURFACE ( 'NONE', #76328, 0.09999999999999982514, 0.003490658503988666988 ) ;
#47096=CIRCLE ( 'NONE', #95113, 0.06509327318403745899 ) ;
#47097=DIRECTION ( 'NONE',  ( 0.000000000000000000, 1.000000000000000000, 0.000000000000000000 ) ) ;
#47099=ORIENTED_EDGE ( 'NONE', *, *, #100441, .F. ) ;
#47100=ORIENTED_EDGE ( 'NONE', *, *, #76978, .F. ) ;
#47101=CARTESIAN_POINT ( 'NONE',  ( -7.700000000000016165, 12.50000000000000000, -3.918623584224389056 ) ) ;
#47102=CARTESIAN_POINT ( 'NONE',  ( 12.49999999999990052, 2.500000000000000000, 0.6928203230275494784 ) ) ;
#47103=CARTESIAN_POINT ( 'NONE',  ( 12.69999999999990159, 2.500000000000000000, 4.776537180435972196 ) ) ;
#47104=CONICAL_SURFACE ( 'NONE', #128689, 0.1000000000000002554, 0.003490658503988666988 ) ;
#47105=DIRECTION ( 'NONE',  ( 0.000000000000000000, 1.000000000000000000, 0.000000000000000000 ) ) ;
#47106=VECTOR ( 'NONE', #20161, 1000.000000000000000 ) ;
#47107=CIRCLE ( 'NONE', #72245, 0.06509327318403745899 ) ;
#47109=CARTESIAN_POINT ( 'NONE',  ( 4.799999999999934097, 12.50000000000000000, 4.611443907251934426 ) ) ;
#47110=LINE ( 'NONE', #35985, #50959 ) ;
#47111=ORIENTED_EDGE ( 'NONE', *, *, #82872, .F. ) ;
#47112=DIRECTION ( 'NONE',  ( 0.000000000000000000, -0.000000000000000000, 1.000000000000000000 ) ) ;
#47113=AXIS2_PLACEMENT_3D ( 'NONE', #127307, #67718, #45525 ) ;
#47114=CARTESIAN_POINT ( 'NONE',  ( 3.349999999999945466, 12.50000000000000000, -2.792790559304616504 ) ) ;
#47115=AXIS2_PLACEMENT_3D ( 'NONE', #60001, #11516, #60638 ) ;
#47117=VERTEX_POINT ( 'NONE', #24933 ) ;
#47118=EDGE_LOOP ( 'NONE', ( #50988, #72353 ) ) ;
#47119=ORIENTED_EDGE ( 'NONE', *, *, #126252, .F. ) ;
#47120=FACE_OUTER_BOUND ( 'NONE', #41443, .T. ) ;
#47121=DIRECTION ( 'NONE',  ( 0.000000000000000000, 0.000000000000000000, 1.000000000000000000 ) ) ;
#47122=ORIENTED_EDGE ( 'NONE', *, *, #30073, .F. ) ;
#47123=LINE ( 'NONE', #15694, #104921 ) ;
#47124=EDGE_CURVE ( 'NONE', #81821, #98256, #112625, .T. ) ;
#47125=CARTESIAN_POINT ( 'NONE',  ( 17.50000000000000000, 2.750000000000000000, -3.432456362931489036 ) ) ;
#47126=DIRECTION ( 'NONE',  ( 0.000000000000000000, 1.000000000000000000, 0.000000000000000000 ) ) ;
#47127=ORIENTED_EDGE ( 'NONE', *, *, #112971, .F. ) ;
#47128=CARTESIAN_POINT ( 'NONE',  ( -2.499999999999996447, 12.50000000000000000, 4.330127018922196314 ) ) ;
#47129=AXIS2_PLACEMENT_3D ( 'NONE', #19667, #110615, #88380 ) ;
#47130=CARTESIAN_POINT ( 'NONE',  ( 5.849999999999932143, 2.500000000000000000, 2.165063509461097713 ) ) ;
#47132=ORIENTED_EDGE ( 'NONE', *, *, #95567, .F. ) ;
#47133=EDGE_LOOP ( 'NONE', ( #15212, #109130, #29364, #112607 ) ) ;
#47134=VERTEX_POINT ( 'NONE', #96231 ) ;
#47135=PLANE ( 'NONE',  #15404 ) ;
#47136=VECTOR ( 'NONE', #107401, 1000.000000000000000 ) ;
#47137=FACE_OUTER_BOUND ( 'NONE', #43366, .T. ) ;
#47139=DIRECTION ( 'NONE',  ( 0.000000000000000000, 0.000000000000000000, 1.000000000000000000 ) ) ;
#47140=DIRECTION ( 'NONE',  ( -0.000000000000000000, 1.000000000000000000, -0.000000000000000000 ) ) ;
#47141=DIRECTION ( 'NONE',  ( 0.000000000000000000, 0.000000000000000000, -1.000000000000000000 ) ) ;
#47142=LINE ( 'NONE', #74656, #121422 ) ;
#47143=AXIS2_PLACEMENT_3D ( 'NONE', #40726, #19779, #121189 ) ;
#47144=ORIENTED_EDGE ( 'NONE', *, *, #79134, .F. ) ;
#47145=CARTESIAN_POINT ( 'NONE',  ( 8.949999999999915801, 12.50000000000000000, -1.818653347947326138 ) ) ;
#47146=VECTOR ( 'NONE', #4995, 1000.000000000000000 ) ;
#47147=EDGE_LOOP ( 'NONE', ( #20605, #56954, #17708, #52181 ) ) ;
#47148=ORIENTED_EDGE ( 'NONE', *, *, #96543, .F. ) ;
#47149=VERTEX_POINT ( 'NONE', #106070 ) ;
#47150=CARTESIAN_POINT ( 'NONE',  ( 4.999999999999971578, 2.500000000000000000, -2.276824562219559311E-15 ) ) ;
#47151=FACE_BOUND ( 'NONE', #34900, .T. ) ;
#47152=DIRECTION ( 'NONE',  ( 0.000000000000000000, 0.000000000000000000, -1.000000000000000000 ) ) ;
#47153=DIRECTION ( 'NONE',  ( 0.000000000000000000, -0.000000000000000000, 1.000000000000000000 ) ) ;
#47154=CARTESIAN_POINT ( 'NONE',  ( 3.299999999999944755, 2.500000000000000000, -4.330127018922201643 ) ) ;
#47155=EDGE_CURVE ( 'NONE', #15933, #100718, #29004, .T. ) ;
#47156=AXIS2_PLACEMENT_3D ( 'NONE', #63102, #84021, #93856 ) ;
#47157=CONICAL_SURFACE ( 'NONE', #126578, 0.09999999999999982514, 0.003490658503988666988 ) ;
#47158=ORIENTED_EDGE ( 'NONE', *, *, #52007, .T. ) ;
#47159=DIRECTION ( 'NONE',  ( 0.000000000000000000, 0.000000000000000000, -1.000000000000000000 ) ) ;
#47161=CARTESIAN_POINT ( 'NONE',  ( -0.4000000000000339950, 2.500000000000000000, 0.6928203230275518099 ) ) ;
#47162=CARTESIAN_POINT ( 'NONE',  ( 4.149999999999939959, 2.500000000000000000, 2.857883832488649301 ) ) ;
#47163=VERTEX_POINT ( 'NONE', #46492 ) ;
#47164=ADVANCED_FACE ( 'NONE', ( #38645 ), #98222, .T. ) ;
#47165=PLANE ( 'NONE',  #115912 ) ;
#47166=LINE ( 'NONE', #7867, #37006 ) ;
#47167=CIRCLE ( 'NONE', #120329, 0.06509327318403745899 ) ;
#47168=ORIENTED_EDGE ( 'NONE', *, *, #59727, .F. ) ;
#47169=EDGE_CURVE ( 'NONE', #37316, #59852, #79471, .T. ) ;
#47170=CARTESIAN_POINT ( 'NONE',  ( -9.150000000000011013, 2.500000000000000000, -5.802370205355744659 ) ) ;
#47171=FACE_OUTER_BOUND ( 'NONE', #102773, .T. ) ;
#47172=ADVANCED_FACE ( 'NONE', ( #107996 ), #127007, .T. ) ;
#47173=CIRCLE ( 'NONE', #126597, 0.1000000000000002554 ) ;
#47174=FACE_BOUND ( 'NONE', #80759, .T. ) ;
#47175=DIRECTION ( 'NONE',  ( -0.000000000000000000, 1.000000000000000000, -0.000000000000000000 ) ) ;
#47176=CIRCLE ( 'NONE', #42995, 0.06509327318403745899 ) ;
#47177=EDGE_LOOP ( 'NONE', ( #31229, #123086 ) ) ;
#47178=DIRECTION ( 'NONE',  ( -0.000000000000000000, -1.000000000000000000, -0.000000000000000000 ) ) ;
#47179=EDGE_CURVE ( 'NONE', #64350, #101033, #58544, .T. ) ;
#47180=CONICAL_SURFACE ( 'NONE', #111926, 0.1000000000000002554, 0.003490658503988666988 ) ;
#47181=EDGE_LOOP ( 'NONE', ( #19351, #38847, #91971, #65506 ) ) ;
#47182=ORIENTED_EDGE ( 'NONE', *, *, #9351, .F. ) ;
#47183=CARTESIAN_POINT ( 'NONE',  ( 6.899999999999928413, 2.500000000000000000, 4.576537180435972019 ) ) ;
#47184=EDGE_CURVE ( 'NONE', #63096, #907, #46016, .T. ) ;
#47186=ORIENTED_EDGE ( 'NONE', *, *, #110364, .T. ) ;
#47189=DIRECTION ( 'NONE',  ( 0.000000000000000000, 0.000000000000000000, 1.000000000000000000 ) ) ;
#47190=CONICAL_SURFACE ( 'NONE', #114087, 0.1000000000000002554, 0.003490658503988666988 ) ;
#47194=VERTEX_POINT ( 'NONE', #36700 ) ;
#47195=AXIS2_PLACEMENT_3D ( 'NONE', #10038, #858, #91173 ) ;
#47196=DIRECTION ( 'NONE',  ( 0.000000000000000000, 1.000000000000000000, 0.000000000000000000 ) ) ;
#47197=CARTESIAN_POINT ( 'NONE',  ( 3.099999999999945466, 12.50000000000000000, 0.2813168883297361700 ) ) ;
#47198=DIRECTION ( 'NONE',  ( 0.000000000000000000, -0.000000000000000000, 1.000000000000000000 ) ) ;
#47199=CONICAL_SURFACE ( 'NONE', #1127, 0.09999999999999982514, 0.003490658503988666988 ) ;
#47200=DIRECTION ( 'NONE',  ( -0.000000000000000000, 1.000000000000000000, -0.000000000000000000 ) ) ;
#47201=VERTEX_POINT ( 'NONE', #76612 ) ;
#47202=DIRECTION ( 'NONE',  ( 0.000000000000000000, 0.000000000000000000, -1.000000000000000000 ) ) ;
#47203=ORIENTED_EDGE ( 'NONE', *, *, #113241, .F. ) ;
#47204=DIRECTION ( 'NONE',  ( 0.000000000000000000, -0.000000000000000000, 1.000000000000000000 ) ) ;
#47205=CARTESIAN_POINT ( 'NONE',  ( 0.8499999999999550138, 2.500000000000000000, -5.802370205355749988 ) ) ;
#47206=ORIENTED_EDGE ( 'NONE', *, *, #72453, .F. ) ;
#47207=PLANE ( 'NONE',  #88765 ) ;
#47208=DIRECTION ( 'NONE',  ( 0.000000000000000000, 1.000000000000000000, 0.000000000000000000 ) ) ;
#47209=EDGE_CURVE ( 'NONE', #48633, #69160, #47802, .T. ) ;
#47210=DIRECTION ( 'NONE',  ( 0.000000000000000000, 0.000000000000000000, 1.000000000000000000 ) ) ;
#47211=CARTESIAN_POINT ( 'NONE',  ( 9.799999999999917222, 12.50000000000000000, 0.3464101615137735735 ) ) ;
#47212=ORIENTED_EDGE ( 'NONE', *, *, #47531, .F. ) ;
#47213=DIRECTION ( 'NONE',  ( 0.000000000000000000, 1.000000000000000000, 0.000000000000000000 ) ) ;
#47214=CARTESIAN_POINT ( 'NONE',  ( -9.800000000000007816, 12.50000000000000000, -3.983716857408421852 ) ) ;
#47216=DIRECTION ( 'NONE',  ( 0.000000000000000000, 0.000000000000000000, -1.000000000000000000 ) ) ;
#47217=AXIS2_PLACEMENT_3D ( 'NONE', #43193, #13695, #123028 ) ;
#47218=DIRECTION ( 'NONE',  ( 0.000000000000000000, -0.000000000000000000, 1.000000000000000000 ) ) ;
#47219=EDGE_CURVE ( 'NONE', #20030, #123959, #62743, .T. ) ;
#47220=EDGE_LOOP ( 'NONE', ( #17744, #96005 ) ) ;
#47221=ORIENTED_EDGE ( 'NONE', *, *, #45289, .F. ) ;
#47222=CARTESIAN_POINT ( 'NONE',  ( -6.900000000000015454, 12.50000000000000000, 3.983716857408420076 ) ) ;
#47223=ORIENTED_EDGE ( 'NONE', *, *, #7568, .F. ) ;
#47224=CARTESIAN_POINT ( 'NONE',  ( -0.6500000000000403233, 2.500000000000000000, 1.718653347947321386 ) ) ;
#47225=EDGE_CURVE ( 'NONE', #88700, #31372, #23020, .T. ) ;
#47226=ORIENTED_EDGE ( 'NONE', *, *, #20613, .T. ) ;
#47227=ORIENTED_EDGE ( 'NONE', *, *, #101355, .T. ) ;
#47228=CIRCLE ( 'NONE', #120383, 0.1000000000000000472 ) ;
#47229=EDGE_LOOP ( 'NONE', ( #32183, #64837, #24363, #51894 ) ) ;
#47230=EDGE_CURVE ( 'NONE', #54992, #48724, #64775, .T. ) ;
#47231=CARTESIAN_POINT ( 'NONE',  ( 13.54999999999989591, 12.50000000000000000, -1.753560074763288679 ) ) ;
#47232=CIRCLE ( 'NONE', #49388, 0.06509327318403745899 ) ;
#47233=EDGE_CURVE ( 'NONE', #45762, #39409, #102158, .T. ) ;
#47234=VECTOR ( 'NONE', #55233, 1000.000000000000000 ) ;
#47235=DIRECTION ( 'NONE',  ( 0.000000000000000000, 0.000000000000000000, 1.000000000000000000 ) ) ;
#47236=DIRECTION ( 'NONE',  ( 0.000000000000000000, 1.000000000000000000, 0.000000000000000000 ) ) ;
#47238=EDGE_CURVE ( 'NONE', #35493, #88394, #24, .T. ) ;
#47239=DIRECTION ( 'NONE',  ( 0.000000000000000000, 0.000000000000000000, 1.000000000000000000 ) ) ;
#47240=DIRECTION ( 'NONE',  ( 0.000000000000000000, 0.000000000000000000, 1.000000000000000000 ) ) ;
#47241=DIRECTION ( 'NONE',  ( 0.000000000000000000, 0.000000000000000000, 1.000000000000000000 ) ) ;
#47242=ORIENTED_EDGE ( 'NONE', *, *, #68957, .T. ) ;
#47243=DIRECTION ( 'NONE',  ( 0.000000000000000000, 0.000000000000000000, 1.000000000000000000 ) ) ;
#47244=EDGE_CURVE ( 'NONE', #67980, #16778, #35270, .T. ) ;
#47245=ORIENTED_EDGE ( 'NONE', *, *, #17769, .F. ) ;
#47246=AXIS2_PLACEMENT_3D ( 'NONE', #35400, #37342, #104749 ) ;
#47247=ADVANCED_FACE ( 'NONE', ( #27482 ), #91692, .T. ) ;
#47248=EDGE_LOOP ( 'NONE', ( #53024, #85382 ) ) ;
#47249=VERTEX_POINT ( 'NONE', #8491 ) ;
#47250=ORIENTED_EDGE ( 'NONE', *, *, #24422, .T. ) ;
#47251=CONICAL_SURFACE ( 'NONE', #49317, 0.1000000000000002554, 0.003490658503988666988 ) ;
#47252=CONICAL_SURFACE ( 'NONE', #53503, 0.1000000000000002554, 0.003490658503988666988 ) ;
#47253=CARTESIAN_POINT ( 'NONE',  ( 10.39999999999991509, 2.500000000000000000, 0.6928203230275494784 ) ) ;
#47254=EDGE_LOOP ( 'NONE', ( #8152, #78123 ) ) ;
#47255=VERTEX_POINT ( 'NONE', #28809 ) ;
#47256=DIRECTION ( 'NONE',  ( -0.000000000000000000, 1.000000000000000000, -0.000000000000000000 ) ) ;
#47258=DIRECTION ( 'NONE',  ( 0.000000000000000000, 1.000000000000000000, 0.000000000000000000 ) ) ;
#47259=AXIS2_PLACEMENT_3D ( 'NONE', #16420, #95659, #113359 ) ;
#47260=DIRECTION ( 'NONE',  ( 0.000000000000000000, 0.000000000000000000, 1.000000000000000000 ) ) ;
#47261=DIRECTION ( 'NONE',  ( -0.000000000000000000, -1.000000000000000000, -0.000000000000000000 ) ) ;
#47262=DIRECTION ( 'NONE',  ( -0.000000000000000000, -1.000000000000000000, -0.000000000000000000 ) ) ;
#47263=ORIENTED_EDGE ( 'NONE', *, *, #92304, .T. ) ;
#47264=FACE_OUTER_BOUND ( 'NONE', #77693, .T. ) ;
#47265=VERTEX_POINT ( 'NONE', #68713 ) ;
#47266=CARTESIAN_POINT ( 'NONE',  ( -9.150000000000011013, 12.50000000000000000, -5.802370205355744659 ) ) ;
#47267=VERTEX_POINT ( 'NONE', #108640 ) ;
#47268=FACE_OUTER_BOUND ( 'NONE', #62958, .T. ) ;
#47270=ORIENTED_EDGE ( 'NONE', *, *, #45747, .T. ) ;
#47271=CARTESIAN_POINT ( 'NONE',  ( -2.050000000000032685, 2.500000000000000000, -2.265063509461101798 ) ) ;
#47272=LINE ( 'NONE', #5396, #21357 ) ;
#47273=CIRCLE ( 'NONE', #76512, 0.06509327318403745899 ) ;
#47274=DIRECTION ( 'NONE',  ( 0.000000000000000000, 1.000000000000000000, 0.000000000000000000 ) ) ;
#47275=EDGE_CURVE ( 'NONE', #81286, #80090, #9155, .T. ) ;
#47276=CIRCLE ( 'NONE', #55665, 0.06509327318403741736 ) ;
#47277=FACE_OUTER_BOUND ( 'NONE', #115545, .T. ) ;
#47278=FACE_OUTER_BOUND ( 'NONE', #42903, .T. ) ;
#47279=ORIENTED_EDGE ( 'NONE', *, *, #35470, .F. ) ;
#47280=DIRECTION ( 'NONE',  ( -0.000000000000000000, -1.000000000000000000, -0.000000000000000000 ) ) ;
#47281=DIRECTION ( 'NONE',  ( 0.000000000000000000, 0.000000000000000000, 1.000000000000000000 ) ) ;
#47282=DIRECTION ( 'NONE',  ( 0.000000000000000000, -0.000000000000000000, 1.000000000000000000 ) ) ;
#47283=FACE_OUTER_BOUND ( 'NONE', #91441, .T. ) ;
#47284=CONICAL_SURFACE ( 'NONE', #120434, 0.1000000000000000472, 0.003490658503988666988 ) ;
#47285=AXIS2_PLACEMENT_3D ( 'NONE', #21404, #22073, #2387 ) ;
#47286=DIRECTION ( 'NONE',  ( -0.000000000000000000, 1.000000000000000000, -0.000000000000000000 ) ) ;
#47287=EDGE_CURVE ( 'NONE', #120157, #32665, #68695, .T. ) ;
#47288=ORIENTED_EDGE ( 'NONE', *, *, #19, .T. ) ;
#47289=ORIENTED_EDGE ( 'NONE', *, *, #27353, .T. ) ;
#47290=CARTESIAN_POINT ( 'NONE',  ( -1.050000000000038680, 2.500000000000000000, 6.841600689897072485 ) ) ;
#47291=EDGE_LOOP ( 'NONE', ( #97792, #33771, #37740, #77419 ) ) ;
#47292=CARTESIAN_POINT ( 'NONE',  ( 5.849999999999935696, 12.50000000000000000, -7.122917578226816815 ) ) ;
#47293=CARTESIAN_POINT ( 'NONE',  ( 7.499999999999927169, 2.500000000000000000, 3.637306695894644726 ) ) ;
#47294=VECTOR ( 'NONE', #115964, 1000.000000000000000 ) ;
#47295=VERTEX_POINT ( 'NONE', #31393 ) ;
#47297=FACE_OUTER_BOUND ( 'NONE', #3111, .T. ) ;
#47298=DIRECTION ( 'NONE',  ( -4.274815082592931898E-19, -0.9999939076577903929, -0.003490651415223739937 ) ) ;
#47299=DIRECTION ( 'NONE',  ( 0.000000000000000000, 0.000000000000000000, -1.000000000000000000 ) ) ;
#47300=ORIENTED_EDGE ( 'NONE', *, *, #51693, .T. ) ;
#47301=CARTESIAN_POINT ( 'NONE',  ( -9.999999999999969802, 2.500000000000000000, 4.230127018922196669 ) ) ;
#47303=VERTEX_POINT ( 'NONE', #90944 ) ;
#47304=DIRECTION ( 'NONE',  ( 0.000000000000000000, 1.000000000000000000, 0.000000000000000000 ) ) ;
#47305=AXIS2_PLACEMENT_3D ( 'NONE', #111086, #111763, #43050 ) ;
#47306=DIRECTION ( 'NONE',  ( 0.000000000000000000, -0.9999939076577903929, 0.003490651415223739937 ) ) ;
#47307=DIRECTION ( 'NONE',  ( 0.000000000000000000, -0.000000000000000000, 1.000000000000000000 ) ) ;
#47308=ORIENTED_EDGE ( 'NONE', *, *, #54442, .T. ) ;
#47309=FACE_OUTER_BOUND ( 'NONE', #99359, .T. ) ;
#47310=CIRCLE ( 'NONE', #34806, 0.09999999999999999167 ) ;
#47311=EDGE_LOOP ( 'NONE', ( #2077, #75655, #23505, #30457 ) ) ;
#47312=CARTESIAN_POINT ( 'NONE',  ( -5.400000000000019895, 12.50000000000000000, 3.637306695894644726 ) ) ;
#47313=FACE_OUTER_BOUND ( 'NONE', #17139, .T. ) ;
#47315=DIRECTION ( 'NONE',  ( 0.000000000000000000, 1.000000000000000000, 0.000000000000000000 ) ) ;
#47316=VECTOR ( 'NONE', #108177, 1000.000000000000000 ) ;
#47317=ORIENTED_EDGE ( 'NONE', *, *, #19884, .F. ) ;
#47318=EDGE_CURVE ( 'NONE', #86156, #37898, #125144, .T. ) ;
#47319=LINE ( 'NONE', #118623, #63519 ) ;
#47320=CIRCLE ( 'NONE', #107955, 0.06509327318403743123 ) ;
#47321=DIRECTION ( 'NONE',  ( 0.000000000000000000, -0.000000000000000000, 1.000000000000000000 ) ) ;
#47322=VERTEX_POINT ( 'NONE', #50368 ) ;
#47323=EDGE_CURVE ( 'NONE', #92653, #72025, #62461, .T. ) ;
#47324=CARTESIAN_POINT ( 'NONE',  ( -10.20000000000000639, 2.500000000000000000, -4.083716857408422385 ) ) ;
#47325=ADVANCED_FACE ( 'NONE', ( #32044 ), #102250, .T. ) ;
#47326=VERTEX_POINT ( 'NONE', #100122 ) ;
#47327=FACE_OUTER_BOUND ( 'NONE', #104754, .T. ) ;
#47328=VECTOR ( 'NONE', #67916, 1000.000000000000000 ) ;
#47329=AXIS2_PLACEMENT_3D ( 'NONE', #39204, #109856, #20829 ) ;
#47330=AXIS2_PLACEMENT_3D ( 'NONE', #7906, #128362, #127688 ) ;
#47331=ORIENTED_EDGE ( 'NONE', *, *, #46927, .T. ) ;
#47332=DIRECTION ( 'NONE',  ( -0.000000000000000000, -1.000000000000000000, -0.000000000000000000 ) ) ;
#47333=DIRECTION ( 'NONE',  ( -4.274815082592931898E-19, -0.9999939076577903929, -0.003490651415223739937 ) ) ;
#47334=EDGE_CURVE ( 'NONE', #71492, #109003, #70022, .T. ) ;
#47335=EDGE_CURVE ( 'NONE', #702, #89145, #6079, .T. ) ;
#47336=ORIENTED_EDGE ( 'NONE', *, *, #11686, .F. ) ;
#47337=ORIENTED_EDGE ( 'NONE', *, *, #4285, .T. ) ;
#47338=EDGE_CURVE ( 'NONE', #109850, #100401, #129375, .T. ) ;
#47339=LINE ( 'NONE', #106875, #1720 ) ;
#47340=CARTESIAN_POINT ( 'NONE',  ( 6.049999999999932321, 2.500000000000000000, -1.818653347947326138 ) ) ;
#47341=VERTEX_POINT ( 'NONE', #59581 ) ;
#47342=LINE ( 'NONE', #87239, #21700 ) ;
#47343=CARTESIAN_POINT ( 'NONE',  ( -11.24999999999996270, 12.50000000000000000, 2.165063509461097713 ) ) ;
#47344=DIRECTION ( 'NONE',  ( 0.000000000000000000, 1.000000000000000000, 0.000000000000000000 ) ) ;
#47345=DIRECTION ( 'NONE',  ( 0.000000000000000000, -0.9999939076577903929, 0.003490651415223739937 ) ) ;
#47346=DIRECTION ( 'NONE',  ( -0.000000000000000000, 1.000000000000000000, -0.000000000000000000 ) ) ;
#47347=DIRECTION ( 'NONE',  ( 0.000000000000000000, 0.000000000000000000, -1.000000000000000000 ) ) ;
#47348=ORIENTED_EDGE ( 'NONE', *, *, #2582, .T. ) ;
#47349=ORIENTED_EDGE ( 'NONE', *, *, #83461, .T. ) ;
#47350=ORIENTED_EDGE ( 'NONE', *, *, #82506, .T. ) ;
#47351=ORIENTED_EDGE ( 'NONE', *, *, #80209, .F. ) ;
#47352=PLANE ( 'NONE',  #66240 ) ;
#47353=CARTESIAN_POINT ( 'NONE',  ( -13.74999999999998934, 12.50000000000000000, -1.472243186433547901 ) ) ;
#47354=LINE ( 'NONE', #127210, #92864 ) ;
#47355=ORIENTED_EDGE ( 'NONE', *, *, #83799, .F. ) ;
#47356=FACE_BOUND ( 'NONE', #69636, .T. ) ;
#47357=DIRECTION ( 'NONE',  ( 0.000000000000000000, 0.000000000000000000, 1.000000000000000000 ) ) ;
#47358=DIRECTION ( 'NONE',  ( 0.000000000000000000, 1.000000000000000000, 0.000000000000000000 ) ) ;
#47359=DIRECTION ( 'NONE',  ( 0.000000000000000000, -0.000000000000000000, 1.000000000000000000 ) ) ;
#47360=CONICAL_SURFACE ( 'NONE', #39067, 0.09999999999999999167, 0.003490658503988666988 ) ;
#47361=LINE ( 'NONE', #27703, #99392 ) ;
#47362=CARTESIAN_POINT ( 'NONE',  ( -12.89999999999999147, 2.500000000000000000, 1.843143693225357538E-15 ) ) ;
#47363=CARTESIAN_POINT ( 'NONE',  ( -2.700000000000030820, 2.500000000000000000, 0.3464101615137735735 ) ) ;
#47364=CARTESIAN_POINT ( 'NONE',  ( 1.649999999999951061, 2.500000000000000000, -6.495190528383302464 ) ) ;
#47365=LINE ( 'NONE', #29026, #91042 ) ;
#47366=DIRECTION ( 'NONE',  ( -0.000000000000000000, 1.000000000000000000, -0.000000000000000000 ) ) ;
#47367=DIRECTION ( 'NONE',  ( 0.000000000000000000, 0.000000000000000000, -1.000000000000000000 ) ) ;
#47368=AXIS2_PLACEMENT_3D ( 'NONE', #21703, #91721, #19085 ) ;
#47369=CIRCLE ( 'NONE', #20266, 0.1000000000000000472 ) ;
#47370=EDGE_LOOP ( 'NONE', ( #34859, #95387, #14680, #28017 ) ) ;
#47371=ORIENTED_EDGE ( 'NONE', *, *, #118115, .T. ) ;
#47372=ORIENTED_EDGE ( 'NONE', *, *, #128245, .F. ) ;
#47373=ORIENTED_EDGE ( 'NONE', *, *, #80724, .F. ) ;
#47374=LINE ( 'NONE', #39512, #60182 ) ;
#47375=ADVANCED_FACE ( 'NONE', ( #1271 ), #41636, .T. ) ;
#47376=DIRECTION ( 'NONE',  ( 0.000000000000000000, 1.000000000000000000, 0.000000000000000000 ) ) ;
#47377=EDGE_CURVE ( 'NONE', #87449, #113705, #1906, .T. ) ;
#47378=VERTEX_POINT ( 'NONE', #30757 ) ;
#47379=ORIENTED_EDGE ( 'NONE', *, *, #70974, .T. ) ;
#47380=ORIENTED_EDGE ( 'NONE', *, *, #55927, .T. ) ;
#47381=EDGE_CURVE ( 'NONE', #19267, #82725, #79827, .T. ) ;
#47382=DIRECTION ( 'NONE',  ( 0.000000000000000000, 1.000000000000000000, 0.000000000000000000 ) ) ;
#47383=AXIS2_PLACEMENT_3D ( 'NONE', #100242, #121162, #41336 ) ;
#47384=AXIS2_PLACEMENT_3D ( 'NONE', #45881, #125697, #53756 ) ;
#47385=AXIS2_PLACEMENT_3D ( 'NONE', #87625, #85698, #75237 ) ;
#47386=DIRECTION ( 'NONE',  ( 0.000000000000000000, 1.000000000000000000, 0.000000000000000000 ) ) ;
#47387=CARTESIAN_POINT ( 'NONE',  ( -12.89999999999999147, 12.50000000000000000, 0.06509327318403926310 ) ) ;
#47388=EDGE_CURVE ( 'NONE', #58176, #116703, #52083, .T. ) ;
#47389=CARTESIAN_POINT ( 'NONE',  ( 6.899999999999928413, 2.500000000000000000, -4.576537180435977348 ) ) ;
#47390=ADVANCED_FACE ( 'NONE', ( #49747 ), #111205, .T. ) ;
#47391=CARTESIAN_POINT ( 'NONE',  ( -2.300000000000033573, 2.500000000000000000, 0.2464101615137735679 ) ) ;
#47392=DIRECTION ( 'NONE',  ( 0.000000000000000000, 1.000000000000000000, 0.000000000000000000 ) ) ;
#47393=ORIENTED_EDGE ( 'NONE', *, *, #113680, .T. ) ;
#47394=DIRECTION ( 'NONE',  ( 0.000000000000000000, 0.000000000000000000, -1.000000000000000000 ) ) ;
#47395=ADVANCED_FACE ( 'NONE', ( #111877 ), #114753, .T. ) ;
#47396=ORIENTED_EDGE ( 'NONE', *, *, #124057, .F. ) ;
#47397=EDGE_CURVE ( 'NONE', #44028, #114232, #52307, .T. ) ;
#47398=ORIENTED_EDGE ( 'NONE', *, *, #54716, .T. ) ;
#47399=ORIENTED_EDGE ( 'NONE', *, *, #87683, .F. ) ;
#47400=PLANE ( 'NONE',  #96428 ) ;
#47401=ORIENTED_EDGE ( 'NONE', *, *, #55940, .T. ) ;
#47402=AXIS2_PLACEMENT_3D ( 'NONE', #13546, #71844, #3731 ) ;
#47403=ORIENTED_EDGE ( 'NONE', *, *, #54719, .T. ) ;
#47404=ADVANCED_FACE ( 'NONE', ( #100742 ), #12375, .T. ) ;
#47405=VECTOR ( 'NONE', #68278, 1000.000000000000000 ) ;
#47406=DIRECTION ( 'NONE',  ( 0.000000000000000000, 1.000000000000000000, 0.000000000000000000 ) ) ;
#47407=CARTESIAN_POINT ( 'NONE',  ( -1.050000000000037348, 12.50000000000000000, -6.841600689897078702 ) ) ;
#47408=DIRECTION ( 'NONE',  ( -4.274815082592931898E-19, -0.9999939076577903929, -0.003490651415223739937 ) ) ;
#47409=CIRCLE ( 'NONE', #105883, 0.06509327318403745899 ) ;
#47410=CARTESIAN_POINT ( 'NONE',  ( -11.89999999999999680, 12.50000000000000000, -0.3464101615137741841 ) ) ;
#47411=CARTESIAN_POINT ( 'NONE',  ( 0.3999999999999555023, 2.500000000000000000, 4.330127018922196314 ) ) ;
#47412=VECTOR ( 'NONE', #114316, 1000.000000000000000 ) ;
#47413=VERTEX_POINT ( 'NONE', #20267 ) ;
#47414=CARTESIAN_POINT ( 'NONE',  ( -14.39999999999998614, 2.500000000000000000, 0.3464101615137758494 ) ) ;
#47416=EDGE_LOOP ( 'NONE', ( #122073, #63840, #34114, #65978 ) ) ;
#47417=AXIS2_PLACEMENT_3D ( 'NONE', #109, #30250, #59713 ) ;
#47419=VERTEX_POINT ( 'NONE', #20911 ) ;
#47420=CARTESIAN_POINT ( 'NONE',  ( 9.999999999999952038, 12.50000000000000000, -2.276824562219559311E-15 ) ) ;
#47421=CARTESIAN_POINT ( 'NONE',  ( -14.99999999999998401, 12.50000000000000000, 0.6928203230275518099 ) ) ;
#47422=VERTEX_POINT ( 'NONE', #60839 ) ;
#47423=DIRECTION ( 'NONE',  ( -0.000000000000000000, 1.000000000000000000, -0.000000000000000000 ) ) ;
#47424=CIRCLE ( 'NONE', #124776, 0.09999999999999982514 ) ;
#47425=CARTESIAN_POINT ( 'NONE',  ( -10.20000000000000462, 2.500000000000000000, -4.776537180435973085 ) ) ;
#47426=ORIENTED_EDGE ( 'NONE', *, *, #111922, .F. ) ;
#47427=AXIS2_PLACEMENT_3D ( 'NONE', #91427, #21391, #71136 ) ;
#47428=AXIS2_PLACEMENT_3D ( 'NONE', #120800, #50776, #13410 ) ;
#47429=CONICAL_SURFACE ( 'NONE', #120573, 0.09999999999999982514, 0.003490658503988666988 ) ;
#47430=CARTESIAN_POINT ( 'NONE',  ( -4.200000000000025935, 2.500000000000000000, 0.09999999999999761857 ) ) ;
#47431=ORIENTED_EDGE ( 'NONE', *, *, #120501, .T. ) ;
#47432=ORIENTED_EDGE ( 'NONE', *, *, #108262, .T. ) ;
#47433=DIRECTION ( 'NONE',  ( -0.000000000000000000, -1.000000000000000000, -0.000000000000000000 ) ) ;
#47434=DIRECTION ( 'NONE',  ( -4.274815082592931898E-19, -0.9999939076577903929, -0.003490651415223739937 ) ) ;
#47436=DIRECTION ( 'NONE',  ( 0.000000000000000000, -0.000000000000000000, 1.000000000000000000 ) ) ;
#47437=DIRECTION ( 'NONE',  ( -0.000000000000000000, -1.000000000000000000, -0.000000000000000000 ) ) ;
#47438=EDGE_CURVE ( 'NONE', #27568, #7845, #37419, .T. ) ;
#47439=LINE ( 'NONE', #105045, #21510 ) ;
#47440=AXIS2_PLACEMENT_3D ( 'NONE', #105151, #3108, #94057 ) ;
#47441=ORIENTED_EDGE ( 'NONE', *, *, #82710, .T. ) ;
#47442=DIRECTION ( 'NONE',  ( -0.000000000000000000, 1.000000000000000000, -0.000000000000000000 ) ) ;
#47443=CARTESIAN_POINT ( 'NONE',  ( 2.299999999999949640, 12.50000000000000000, -0.3464101615137782364 ) ) ;
#47444=EDGE_LOOP ( 'NONE', ( #14111, #43539, #41849, #97835 ) ) ;
#47445=CARTESIAN_POINT ( 'NONE',  ( 12.89999999999989910, 2.500000000000000000, 0.5928203230275495006 ) ) ;
#47446=DIRECTION ( 'NONE',  ( 0.000000000000000000, 0.000000000000000000, -1.000000000000000000 ) ) ;
#47447=CARTESIAN_POINT ( 'NONE',  ( -14.14999999999998614, 12.50000000000000000, 2.099970236277064028 ) ) ;
#47448=FACE_OUTER_BOUND ( 'NONE', #21366, .T. ) ;
#47449=DIRECTION ( 'NONE',  ( 0.000000000000000000, 1.000000000000000000, 0.000000000000000000 ) ) ;
#47450=ORIENTED_EDGE ( 'NONE', *, *, #105256, .F. ) ;
#47451=AXIS2_PLACEMENT_3D ( 'NONE', #34014, #5820, #72658 ) ;
#47452=VECTOR ( 'NONE', #9769, 1000.000000000000000 ) ;
#47453=DIRECTION ( 'NONE',  ( 0.000000000000000000, 0.000000000000000000, 1.000000000000000000 ) ) ;
#47454=DIRECTION ( 'NONE',  ( 0.000000000000000000, 1.000000000000000000, 0.000000000000000000 ) ) ;
#47455=ORIENTED_EDGE ( 'NONE', *, *, #65516, .F. ) ;
#47456=CIRCLE ( 'NONE', #62142, 0.1000000000000002554 ) ;
#47457=AXIS2_PLACEMENT_3D ( 'NONE', #42697, #122521, #72776 ) ;
#47458=CARTESIAN_POINT ( 'NONE',  ( -0.2000000000000408673, 2.500000000000000000, -3.983716857408426293 ) ) ;
#47459=VERTEX_POINT ( 'NONE', #62784 ) ;
#47460=VERTEX_POINT ( 'NONE', #63417 ) ;
#47461=CARTESIAN_POINT ( 'NONE',  ( 7.299999999999927880, 2.500000000000000000, -4.676537180435977881 ) ) ;
#47462=ORIENTED_EDGE ( 'NONE', *, *, #36078, .F. ) ;
#47463=LINE ( 'NONE', #86067, #57218 ) ;
#47464=LINE ( 'NONE', #128631, #94425 ) ;
#47465=CONICAL_SURFACE ( 'NONE', #120629, 0.1000000000000000472, 0.003490658503988666988 ) ;
#47466=CARTESIAN_POINT ( 'NONE',  ( 14.59999999999989484, 2.500000000000000000, -0.6928203230275541413 ) ) ;
#47467=ORIENTED_EDGE ( 'NONE', *, *, #13914, .T. ) ;
#47468=VECTOR ( 'NONE', #21253, 1000.000000000000000 ) ;
#47469=ADVANCED_FACE ( 'NONE', ( #93522 ), #56269, .T. ) ;
#47470=FACE_BOUND ( 'NONE', #109332, .T. ) ;
#47471=DIRECTION ( 'NONE',  ( -0.000000000000000000, 1.000000000000000000, -0.000000000000000000 ) ) ;
#47472=ORIENTED_EDGE ( 'NONE', *, *, #49020, .F. ) ;
#47473=DIRECTION ( 'NONE',  ( 0.000000000000000000, 0.000000000000000000, -1.000000000000000000 ) ) ;
#47474=EDGE_CURVE ( 'NONE', #99703, #20674, #3946, .T. ) ;
#47475=PLANE ( 'NONE',  #113658 ) ;
#47476=EDGE_CURVE ( 'NONE', #24974, #120381, #45822, .T. ) ;
#47477=ORIENTED_EDGE ( 'NONE', *, *, #34546, .F. ) ;
#47478=ORIENTED_EDGE ( 'NONE', *, *, #65946, .T. ) ;
#47479=ORIENTED_EDGE ( 'NONE', *, *, #71138, .T. ) ;
#47480=CARTESIAN_POINT ( 'NONE',  ( -11.89999999999999503, 2.500000000000000000, 4.676537180435972552 ) ) ;
#47481=FACE_OUTER_BOUND ( 'NONE', #66305, .T. ) ;
#47482=EDGE_CURVE ( 'NONE', #87449, #55169, #98035, .T. ) ;
#47483=ADVANCED_FACE ( 'NONE', ( #53606 ), #104616, .T. ) ;
#47484=DIRECTION ( 'NONE',  ( -4.274815082592931898E-19, -0.9999939076577903929, -0.003490651415223739937 ) ) ;
#47485=EDGE_CURVE ( 'NONE', #9662, #11963, #58352, .T. ) ;
#47486=FACE_BOUND ( 'NONE', #20957, .T. ) ;
#47487=ORIENTED_EDGE ( 'NONE', *, *, #129123, .T. ) ;
#47488=EDGE_CURVE ( 'NONE', #3359, #127971, #43797, .T. ) ;
#47489=ADVANCED_FACE ( 'NONE', ( #74529 ), #66633, .T. ) ;
#47490=AXIS2_PLACEMENT_3D ( 'NONE', #79256, #28212, #30157 ) ;
#47491=CARTESIAN_POINT ( 'NONE',  ( 9.399999999999915090, 12.50000000000000000, 4.611443907251934426 ) ) ;
#47492=CARTESIAN_POINT ( 'NONE',  ( 4.799999999999937650, 2.500000000000000000, -0.3464101615137782364 ) ) ;
#47493=AXIS2_PLACEMENT_3D ( 'NONE', #96291, #24988, #104192 ) ;
#47494=VERTEX_POINT ( 'NONE', #52959 ) ;
#47496=CIRCLE ( 'NONE', #14021, 0.09999999999999982514 ) ;
#47497=DIRECTION ( 'NONE',  ( 0.000000000000000000, 0.000000000000000000, -1.000000000000000000 ) ) ;
#47498=CARTESIAN_POINT ( 'NONE',  ( -16.50000000000000000, -1.500000000000000000, 1.734723475976807094E-15 ) ) ;
#47499=EDGE_CURVE ( 'NONE', #18828, #106287, #35357, .T. ) ;
#47500=CARTESIAN_POINT ( 'NONE',  ( -12.29999999999999538, 12.50000000000000000, -4.676537180435976104 ) ) ;
#47501=CIRCLE ( 'NONE', #118586, 0.06509327318403745899 ) ;
#47502=DIRECTION ( 'NONE',  ( -0.000000000000000000, -1.000000000000000000, -0.000000000000000000 ) ) ;
#47503=CONICAL_SURFACE ( 'NONE', #95613, 0.1000000000000002554, 0.003490658503988666988 ) ;
#47504=EDGE_CURVE ( 'NONE', #20024, #91438, #83069, .T. ) ;
#47505=CONICAL_SURFACE ( 'NONE', #74687, 0.09999999999999999167, 0.003490658503988666988 ) ;
#47506=EDGE_LOOP ( 'NONE', ( #92323, #92738 ) ) ;
#47507=EDGE_LOOP ( 'NONE', ( #9380, #17181 ) ) ;
#47508=ORIENTED_EDGE ( 'NONE', *, *, #48818, .F. ) ;
#47509=ORIENTED_EDGE ( 'NONE', *, *, #121380, .F. ) ;
#47510=ORIENTED_EDGE ( 'NONE', *, *, #88894, .F. ) ;
#47512=CARTESIAN_POINT ( 'NONE',  ( 3.349999999999945466, 2.500000000000000000, -6.395190528383301931 ) ) ;
#47513=VECTOR ( 'NONE', #49011, 1000.000000000000000 ) ;
#47514=EDGE_LOOP ( 'NONE', ( #122601, #31726, #115255, #106367 ) ) ;
#47515=FACE_BOUND ( 'NONE', #95875, .T. ) ;
#47516=DIRECTION ( 'NONE',  ( 0.000000000000000000, 1.000000000000000000, 0.000000000000000000 ) ) ;
#47517=CIRCLE ( 'NONE', #120675, 0.06509327318403745899 ) ;
#47518=AXIS2_PLACEMENT_3D ( 'NONE', #57667, #116565, #87107 ) ;
#47519=DIRECTION ( 'NONE',  ( -0.000000000000000000, 1.000000000000000000, -0.000000000000000000 ) ) ;
#47521=DIRECTION ( 'NONE',  ( 0.000000000000000000, 0.000000000000000000, 1.000000000000000000 ) ) ;
#47522=CARTESIAN_POINT ( 'NONE',  ( -10.45000000000000462, 2.500000000000000000, -6.595190528383298556 ) ) ;
#47523=ORIENTED_EDGE ( 'NONE', *, *, #86189, .F. ) ;
#47524=DIRECTION ( 'NONE',  ( 0.000000000000000000, 0.000000000000000000, 1.000000000000000000 ) ) ;
#47525=EDGE_LOOP ( 'NONE', ( #18911, #34923 ) ) ;
#47526=VERTEX_POINT ( 'NONE', #24785 ) ;
#47527=EDGE_LOOP ( 'NONE', ( #114486, #111301 ) ) ;
#47528=DIRECTION ( 'NONE',  ( 0.000000000000000000, 0.000000000000000000, 1.000000000000000000 ) ) ;
#47529=DIRECTION ( 'NONE',  ( 0.000000000000000000, 1.000000000000000000, 0.000000000000000000 ) ) ;
#47530=DIRECTION ( 'NONE',  ( 0.000000000000000000, 0.000000000000000000, 1.000000000000000000 ) ) ;
#47531=EDGE_CURVE ( 'NONE', #79131, #122997, #54129, .T. ) ;
#47532=EDGE_LOOP ( 'NONE', ( #114339, #25189 ) ) ;
#47533=AXIS2_PLACEMENT_3D ( 'NONE', #126237, #44452, #75834 ) ;
#47534=CARTESIAN_POINT ( 'NONE',  ( 16.56576425165006228, 1.499999999999999778, -6.084390597445810123 ) ) ;
#47535=EDGE_CURVE ( 'NONE', #30131, #78082, #25400, .T. ) ;
#47536=FACE_OUTER_BOUND ( 'NONE', #17317, .T. ) ;
#47537=EDGE_CURVE ( 'NONE', #90525, #128150, #33334, .T. ) ;
#47538=DIRECTION ( 'NONE',  ( 0.000000000000000000, -0.000000000000000000, 1.000000000000000000 ) ) ;
#47540=DIRECTION ( 'NONE',  ( 0.000000000000000000, 1.000000000000000000, 0.000000000000000000 ) ) ;
#47542=DIRECTION ( 'NONE',  ( -4.274815082592931898E-19, -0.9999939076577903929, -0.003490651415223739937 ) ) ;
#47543=ADVANCED_FACE ( 'NONE', ( #124917 ), #83382, .T. ) ;
#47544=ORIENTED_EDGE ( 'NONE', *, *, #2286, .T. ) ;
#47545=DIRECTION ( 'NONE',  ( -4.274815082592931898E-19, -0.9999939076577903929, -0.003490651415223739937 ) ) ;
#47546=EDGE_CURVE ( 'NONE', #44909, #113919, #73877, .T. ) ;
#47547=CIRCLE ( 'NONE', #78949, 0.06509327318403741736 ) ;
#47548=EDGE_LOOP ( 'NONE', ( #31247, #69258 ) ) ;
#47549=CIRCLE ( 'NONE', #66309, 0.1000000000000000472 ) ;
#47550=ADVANCED_FACE ( 'NONE', ( #34623 ), #104302, .T. ) ;
#47551=VERTEX_POINT ( 'NONE', #65331 ) ;
#47552=DIRECTION ( 'NONE',  ( -0.000000000000000000, 1.000000000000000000, -0.000000000000000000 ) ) ;
#47553=CARTESIAN_POINT ( 'NONE',  ( 7.899999999999923084, 2.500000000000000000, 0.5928203230275495006 ) ) ;
#47555=ORIENTED_EDGE ( 'NONE', *, *, #106364, .F. ) ;
#47556=ADVANCED_FACE ( 'NONE', ( #105273 ), #68796, .T. ) ;
#47557=AXIS2_PLACEMENT_3D ( 'NONE', #52937, #22206, #113794 ) ;
#47558=AXIS2_PLACEMENT_3D ( 'NONE', #67201, #65944, #107152 ) ;
#47559=VERTEX_POINT ( 'NONE', #8990 ) ;
#47560=CARTESIAN_POINT ( 'NONE',  ( 6.449999999999930012, 12.50000000000000000, -1.753560074763288679 ) ) ;
#47561=CIRCLE ( 'NONE', #120708, 0.06509327318403745899 ) ;
#47562=DIRECTION ( 'NONE',  ( -0.000000000000000000, 1.000000000000000000, -0.000000000000000000 ) ) ;
#47563=CARTESIAN_POINT ( 'NONE',  ( 4.149999999999938183, 2.500000000000000000, 2.265063509461097357 ) ) ;
#47564=ORIENTED_EDGE ( 'NONE', *, *, #38958, .T. ) ;
#47565=EDGE_LOOP ( 'NONE', ( #38008, #62882 ) ) ;
#47566=CARTESIAN_POINT ( 'NONE',  ( -7.300000000000018474, 2.500000000000000000, 0.3464101615137735735 ) ) ;
#47567=CONICAL_SURFACE ( 'NONE', #99793, 0.1000000000000002554, 0.003490658503988666988 ) ;
#47568=ORIENTED_EDGE ( 'NONE', *, *, #63171, .T. ) ;
#47569=DIRECTION ( 'NONE',  ( -0.000000000000000000, 1.000000000000000000, -0.000000000000000000 ) ) ;
#47570=AXIS2_PLACEMENT_3D ( 'NONE', #99025, #127835, #9355 ) ;
#47572=ORIENTED_EDGE ( 'NONE', *, *, #26819, .F. ) ;
#47573=CARTESIAN_POINT ( 'NONE',  ( 14.99999999999989342, 2.500000000000000000, -0.6928203230275541413 ) ) ;
#47574=PLANE ( 'NONE',  #108915 ) ;
#47575=DIRECTION ( 'NONE',  ( 0.000000000000000000, -0.9999939076577903929, 0.003490651415223739937 ) ) ;
#47576=EDGE_CURVE ( 'NONE', #18946, #35145, #125234, .T. ) ;
#47577=CARTESIAN_POINT ( 'NONE',  ( 10.79999999999991367, 2.500000000000000000, -0.1000000000000023925 ) ) ;
#47578=ORIENTED_EDGE ( 'NONE', *, *, #122610, .F. ) ;
#47579=DIRECTION ( 'NONE',  ( -4.274815082592931898E-19, -0.9999939076577903929, -0.003490651415223739937 ) ) ;
#47580=AXIS2_PLACEMENT_3D ( 'NONE', #61858, #51405, #71027 ) ;
#47581=AXIS2_PLACEMENT_3D ( 'NONE', #129013, #118508, #89064 ) ;
#47582=VERTEX_POINT ( 'NONE', #86912 ) ;
#47583=ORIENTED_EDGE ( 'NONE', *, *, #93315, .T. ) ;
#47584=DIRECTION ( 'NONE',  ( 0.000000000000000000, -0.9999939076577903929, 0.003490651415223739937 ) ) ;
#47585=DIRECTION ( 'NONE',  ( 0.000000000000000000, 0.000000000000000000, 1.000000000000000000 ) ) ;
#47586=CARTESIAN_POINT ( 'NONE',  ( 13.94999999999989626, 2.500000000000000000, 2.511473670974873507 ) ) ;
#47587=CARTESIAN_POINT ( 'NONE',  ( -9.150000000000009237, 12.50000000000000000, -1.472243186433550122 ) ) ;
#47588=AXIS2_PLACEMENT_3D ( 'NONE', #31927, #1798, #25153 ) ;
#47589=LINE ( 'NONE', #46281, #48965 ) ;
#47590=AXIS2_PLACEMENT_3D ( 'NONE', #31444, #22278, #1318 ) ;
#47591=CARTESIAN_POINT ( 'NONE',  ( -7.300000000000016698, 2.500000000000000000, -0.3464101615137783474 ) ) ;
#47592=CIRCLE ( 'NONE', #3660, 0.09999999999999982514 ) ;
#47593=DIRECTION ( 'NONE',  ( 0.000000000000000000, -0.9999939076577903929, 0.003490651415223739937 ) ) ;
#47595=DIRECTION ( 'NONE',  ( 0.000000000000000000, 0.000000000000000000, -1.000000000000000000 ) ) ;
#47596=CARTESIAN_POINT ( 'NONE',  ( 9.149999999999918643, 2.500000000000000000, -6.395190528383301931 ) ) ;
#47597=CIRCLE ( 'NONE', #127014, 9.000000000000001776 ) ;
#47598=CONICAL_SURFACE ( 'NONE', #66363, 0.1000000000000002554, 0.003490658503988666988 ) ;
#47599=FACE_OUTER_BOUND ( 'NONE', #104393, .T. ) ;
#47600=AXIS2_PLACEMENT_3D ( 'NONE', #126183, #18152, #36535 ) ;
#47601=ORIENTED_EDGE ( 'NONE', *, *, #12703, .F. ) ;
#47602=DIRECTION ( 'NONE',  ( 0.000000000000000000, 1.000000000000000000, 0.000000000000000000 ) ) ;
#47603=EDGE_CURVE ( 'NONE', #46223, #48711, #116810, .T. ) ;
#47604=DIRECTION ( 'NONE',  ( 0.000000000000000000, 1.000000000000000000, 0.000000000000000000 ) ) ;
#47605=CARTESIAN_POINT ( 'NONE',  ( -3.550000000000027800, 12.50000000000000000, 6.213873640053558134 ) ) ;
#47606=CARTESIAN_POINT ( 'NONE',  ( 9.599999999999914380, 12.50000000000000000, -3.637306695894650055 ) ) ;
#47607=DIRECTION ( 'NONE',  ( -0.000000000000000000, -1.000000000000000000, -0.000000000000000000 ) ) ;
#47608=ORIENTED_EDGE ( 'NONE', *, *, #123324, .F. ) ;
#47609=DIRECTION ( 'NONE',  ( 0.000000000000000000, 0.000000000000000000, 1.000000000000000000 ) ) ;
#47610=CONICAL_SURFACE ( 'NONE', #97777, 0.09999999999999982514, 0.003490658503988666988 ) ;
#47611=AXIS2_PLACEMENT_3D ( 'NONE', #120141, #28535, #69087 ) ;
#47612=CARTESIAN_POINT ( 'NONE',  ( 9.599999999999917932, 12.50000000000000000, -0.6928203230275541413 ) ) ;
#47613=DIRECTION ( 'NONE',  ( 0.000000000000000000, 0.000000000000000000, 1.000000000000000000 ) ) ;
#47615=ORIENTED_EDGE ( 'NONE', *, *, #126756, .F. ) ;
#47616=ORIENTED_EDGE ( 'NONE', *, *, #29198, .T. ) ;
#47617=ORIENTED_EDGE ( 'NONE', *, *, #105248, .T. ) ;
#47618=ORIENTED_EDGE ( 'NONE', *, *, #34042, .T. ) ;
#47619=DIRECTION ( 'NONE',  ( -0.000000000000000000, 1.000000000000000000, -0.000000000000000000 ) ) ;
#47620=CARTESIAN_POINT ( 'NONE',  ( 1.649999999999951505, 2.500000000000000000, -1.372243186433550033 ) ) ;
#47621=CARTESIAN_POINT ( 'NONE',  ( -5.000000000000026645, 2.500000000000000000, -3.737306695894649700 ) ) ;
#47622=CARTESIAN_POINT ( 'NONE',  ( 9.349999999999916156, 12.50000000000000000, -1.883746621131363597 ) ) ;
#47623=ORIENTED_EDGE ( 'NONE', *, *, #65085, .T. ) ;
#47624=EDGE_CURVE ( 'NONE', #40083, #9515, #87554, .T. ) ;
#47625=DIRECTION ( 'NONE',  ( -4.274815082592931898E-19, -0.9999939076577903929, -0.003490651415223739937 ) ) ;
#47626=ORIENTED_EDGE ( 'NONE', *, *, #9831, .T. ) ;
#47627=CARTESIAN_POINT ( 'NONE',  ( 23.85240649352905962, -2.660544618042189224, -4.258220037323775742 ) ) ;
#47628=CARTESIAN_POINT ( 'NONE',  ( 4.149999999999939959, 12.50000000000000000, -2.099970236277064473 ) ) ;
#47630=DIRECTION ( 'NONE',  ( 0.000000000000000000, 0.000000000000000000, 1.000000000000000000 ) ) ;
#47631=CARTESIAN_POINT ( 'NONE',  ( -1.450000000000035483, 2.500000000000000000, 6.148780366869520897 ) ) ;
#47632=ADVANCED_FACE ( 'NONE', ( #75798 ), #108595, .T. ) ;
#47633=ORIENTED_EDGE ( 'NONE', *, *, #78534, .F. ) ;
#47634=CIRCLE ( 'NONE', #37179, 0.1000000000000000472 ) ;
#47635=VERTEX_POINT ( 'NONE', #26717 ) ;
#47636=ORIENTED_EDGE ( 'NONE', *, *, #55513, .F. ) ;
#47637=VERTEX_POINT ( 'NONE', #18818 ) ;
#47638=PLANE ( 'NONE',  #19021 ) ;
#47639=FACE_OUTER_BOUND ( 'NONE', #83791, .T. ) ;
#47640=ADVANCED_FACE ( 'NONE', ( #56158 ), #127387, .T. ) ;
#47641=ADVANCED_FACE ( 'NONE', ( #27333 ), #24968, .T. ) ;
#47642=CARTESIAN_POINT ( 'NONE',  ( -9.350000000000004974, 12.50000000000000000, 6.083687093685483660 ) ) ;
#47643=EDGE_CURVE ( 'NONE', #121018, #128018, #67919, .T. ) ;
#47644=FACE_BOUND ( 'NONE', #22078, .T. ) ;
#47645=ADVANCED_FACE ( 'NONE', ( #96094 ), #67240, .T. ) ;
#47646=DIRECTION ( 'NONE',  ( 0.000000000000000000, 1.000000000000000000, 0.000000000000000000 ) ) ;
#47647=DIRECTION ( 'NONE',  ( 0.000000000000000000, 1.000000000000000000, 0.000000000000000000 ) ) ;
#47648=AXIS2_PLACEMENT_3D ( 'NONE', #43242, #3298, #32134 ) ;
#47650=DIRECTION ( 'NONE',  ( 0.000000000000000000, 0.000000000000000000, -1.000000000000000000 ) ) ;
#47651=AXIS2_PLACEMENT_3D ( 'NONE', #88426, #37423, #107435 ) ;
#47652=AXIS2_PLACEMENT_3D ( 'NONE', #64426, #84714, #22114 ) ;
#47653=ADVANCED_FACE ( 'NONE', ( #17521 ), #38491, .T. ) ;
#47655=CARTESIAN_POINT ( 'NONE',  ( -1.900000000000034994, 12.50000000000000000, -0.2813168883297409439 ) ) ;
#47656=EDGE_CURVE ( 'NONE', #106136, #108138, #112809, .T. ) ;
#47657=DIRECTION ( 'NONE',  ( 0.000000000000000000, -0.000000000000000000, 1.000000000000000000 ) ) ;
#47658=ADVANCED_FACE ( 'NONE', ( #28660 ), #45909, .T. ) ;
#47659=AXIS2_PLACEMENT_3D ( 'NONE', #66808, #8528, #38012 ) ;
#47660=EDGE_CURVE ( 'NONE', #13897, #66518, #79364, .T. ) ;
#47661=FACE_OUTER_BOUND ( 'NONE', #8313, .T. ) ;
#47662=ORIENTED_EDGE ( 'NONE', *, *, #111115, .T. ) ;
#47663=ORIENTED_EDGE ( 'NONE', *, *, #92352, .T. ) ;
#47664=VERTEX_POINT ( 'NONE', #118312 ) ;
#47665=EDGE_LOOP ( 'NONE', ( #108365, #893, #19078, #32263 ) ) ;
#47666=CONICAL_SURFACE ( 'NONE', #89423, 0.1000000000000000472, 0.003490658503988666988 ) ;
#47667=DIRECTION ( 'NONE',  ( -0.000000000000000000, -1.000000000000000000, -0.000000000000000000 ) ) ;
#47668=FACE_BOUND ( 'NONE', #59667, .T. ) ;
#47669=EDGE_CURVE ( 'NONE', #112381, #63537, #77107, .T. ) ;
#47670=CARTESIAN_POINT ( 'NONE',  ( 4.599999999999939249, 2.500000000000000000, -3.537306695894649966 ) ) ;
#47671=AXIS2_PLACEMENT_3D ( 'NONE', #35889, #55537, #93041 ) ;
#47672=STYLED_ITEM ( 'NONE', ( #61731 ), #119481 ) ;
#47673=ORIENTED_EDGE ( 'NONE', *, *, #66214, .T. ) ;
#47674=CARTESIAN_POINT ( 'NONE',  ( -12.89999999999999147, 2.500000000000000000, -0.6928203230275500335 ) ) ;
#47675=CARTESIAN_POINT ( 'NONE',  ( -11.64999999999999858, 2.500000000000000000, -5.802370205355746435 ) ) ;
#47676=FACE_OUTER_BOUND ( 'NONE', #128054, .T. ) ;
#47677=VECTOR ( 'NONE', #11961, 1000.000000000000000 ) ;
#47678=EDGE_LOOP ( 'NONE', ( #55974, #59412 ) ) ;
#47679=CARTESIAN_POINT ( 'NONE',  ( 9.999999999999911182, 2.500000000000000000, -3.637306695894650055 ) ) ;
#47680=AXIS2_PLACEMENT_3D ( 'NONE', #73297, #60904, #41927 ) ;
#47681=CARTESIAN_POINT ( 'NONE',  ( 11.64999999999990443, 2.500000000000000000, -5.802370205355749988 ) ) ;
#47682=AXIS2_PLACEMENT_3D ( 'NONE', #115358, #34922, #35556 ) ;
#47683=ORIENTED_EDGE ( 'NONE', *, *, #35732, .F. ) ;
#47684=DIRECTION ( 'NONE',  ( 0.000000000000000000, -0.9999939076577903929, 0.003490651415223739937 ) ) ;
#47685=CARTESIAN_POINT ( 'NONE',  ( 3.099999999999945466, 12.50000000000000000, -3.983716857408426293 ) ) ;
#47686=AXIS2_PLACEMENT_3D ( 'NONE', #64897, #76670, #95025 ) ;
#47687=AXIS2_PLACEMENT_3D ( 'NONE', #99696, #119971, #78776 ) ;
#47688=ORIENTED_EDGE ( 'NONE', *, *, #106733, .T. ) ;
#47689=CARTESIAN_POINT ( 'NONE',  ( -3.750000000000031086, 12.50000000000000000, -5.867463478539787225 ) ) ;
#47690=DIRECTION ( 'NONE',  ( 0.000000000000000000, 1.000000000000000000, 0.000000000000000000 ) ) ;
#47691=VERTEX_POINT ( 'NONE', #96725 ) ;
#47692=DIRECTION ( 'NONE',  ( 0.000000000000000000, 0.000000000000000000, 1.000000000000000000 ) ) ;
#47693=VERTEX_POINT ( 'NONE', #68561 ) ;
#47694=ORIENTED_EDGE ( 'NONE', *, *, #26652, .F. ) ;
#47695=CIRCLE ( 'NONE', #93659, 0.06509327318403745899 ) ;
#47696=DIRECTION ( 'NONE',  ( 0.000000000000000000, 0.000000000000000000, 1.000000000000000000 ) ) ;
#47697=ORIENTED_EDGE ( 'NONE', *, *, #38969, .T. ) ;
#47698=LINE ( 'NONE', #19509, #47106 ) ;
#47699=FACE_BOUND ( 'NONE', #62110, .T. ) ;
#47700=ADVANCED_FACE ( 'NONE', ( #47009 ), #58119, .T. ) ;
#47701=CIRCLE ( 'NONE', #79099, 0.06509327318403745899 ) ;
#47703=CARTESIAN_POINT ( 'NONE',  ( -14.54999999999998472, 12.50000000000000000, -2.230156782645137170 ) ) ;
#47704=EDGE_CURVE ( 'NONE', #58017, #40065, #8350, .T. ) ;
#47705=ORIENTED_EDGE ( 'NONE', *, *, #77078, .F. ) ;
#47706=DIRECTION ( 'NONE',  ( 0.000000000000000000, 0.000000000000000000, -1.000000000000000000 ) ) ;
#47707=DIRECTION ( 'NONE',  ( -0.000000000000000000, -1.000000000000000000, -0.000000000000000000 ) ) ;
#47708=DIRECTION ( 'NONE',  ( 0.000000000000000000, 1.000000000000000000, 0.000000000000000000 ) ) ;
#47709=DIRECTION ( 'NONE',  ( -0.000000000000000000, 1.000000000000000000, -0.000000000000000000 ) ) ;
#47710=CARTESIAN_POINT ( 'NONE',  ( 10.44999999999991402, 2.500000000000000000, -2.165063509461101710 ) ) ;
#47711=EDGE_CURVE ( 'NONE', #37437, #44623, #89724, .T. ) ;
#47712=VERTEX_POINT ( 'NONE', #31872 ) ;
#47713=ORIENTED_EDGE ( 'NONE', *, *, #72659, .T. ) ;
#47714=FACE_OUTER_BOUND ( 'NONE', #92721, .T. ) ;
#47715=DIRECTION ( 'NONE',  ( 0.000000000000000000, 0.000000000000000000, 1.000000000000000000 ) ) ;
#47717=VERTEX_POINT ( 'NONE', #118956 ) ;
#47718=EDGE_LOOP ( 'NONE', ( #126506, #39989 ) ) ;
#47719=ORIENTED_EDGE ( 'NONE', *, *, #45543, .T. ) ;
#47720=DIRECTION ( 'NONE',  ( 0.000000000000000000, 1.000000000000000000, 0.000000000000000000 ) ) ;
#47721=DIRECTION ( 'NONE',  ( 0.000000000000000000, -0.9999939076577903929, 0.003490651415223739937 ) ) ;
#47722=DIRECTION ( 'NONE',  ( 0.000000000000000000, 0.000000000000000000, 1.000000000000000000 ) ) ;
#47724=LINE ( 'NONE', #127566, #55686 ) ;
#47725=DIRECTION ( 'NONE',  ( 0.000000000000000000, 0.000000000000000000, 1.000000000000000000 ) ) ;
#47726=CIRCLE ( 'NONE', #33070, 0.06509327318403743123 ) ;
#47727=AXIS2_PLACEMENT_3D ( 'NONE', #61569, #32108, #11146 ) ;
#47728=CARTESIAN_POINT ( 'NONE',  ( -13.34999999999999076, 12.50000000000000000, 2.857883832488652853 ) ) ;
#47729=DIRECTION ( 'NONE',  ( 0.000000000000000000, 0.000000000000000000, -1.000000000000000000 ) ) ;
#47730=CARTESIAN_POINT ( 'NONE',  ( 12.49999999999993605, 12.50000000000000000, -2.276824562219559311E-15 ) ) ;
#47731=AXIS2_PLACEMENT_3D ( 'NONE', #73119, #113034, #81639 ) ;
#47732=ORIENTED_EDGE ( 'NONE', *, *, #32557, .F. ) ;
#47733=AXIS2_PLACEMENT_3D ( 'NONE', #121761, #122427, #42589 ) ;
#47734=ORIENTED_EDGE ( 'NONE', *, *, #12351, .F. ) ;
#47735=AXIS2_PLACEMENT_3D ( 'NONE', #122266, #62701, #3766 ) ;
#47736=CARTESIAN_POINT ( 'NONE',  ( -8.100000000000013856, 2.500000000000000000, -0.3464101615137782364 ) ) ;
#47737=ORIENTED_EDGE ( 'NONE', *, *, #109122, .F. ) ;
#47738=ORIENTED_EDGE ( 'NONE', *, *, #52848, .T. ) ;
#47739=PLANE ( 'NONE',  #271 ) ;
#47740=LINE ( 'NONE', #87640, #5136 ) ;
#47741=CARTESIAN_POINT ( 'NONE',  ( -11.04999999999999893, 12.50000000000000000, 1.818653347947321475 ) ) ;
#47742=AXIS2_PLACEMENT_3D ( 'NONE', #91676, #1995, #44411 ) ;
#47743=CARTESIAN_POINT ( 'NONE',  ( -5.850000000000019185, 2.500000000000000000, 2.165063509461097713 ) ) ;
#47744=AXIS2_PLACEMENT_3D ( 'NONE', #22328, #122456, #33438 ) ;
#47745=CARTESIAN_POINT ( 'NONE',  ( 7.699999999999923794, 12.50000000000000000, -3.983716857408426293 ) ) ;
#47746=DIRECTION ( 'NONE',  ( -4.274815082592931898E-19, -0.9999939076577903929, -0.003490651415223739937 ) ) ;
#47747=FACE_OUTER_BOUND ( 'NONE', #89226, .T. ) ;
#47748=ORIENTED_EDGE ( 'NONE', *, *, #44636, .T. ) ;
#47749=CARTESIAN_POINT ( 'NONE',  ( -13.34999999999999076, 2.500000000000000000, -2.857883832488651521 ) ) ;
#47750=LINE ( 'NONE', #16949, #89753 ) ;
#47751=CIRCLE ( 'NONE', #12219, 0.06509327318403745899 ) ;
#47752=EDGE_LOOP ( 'NONE', ( #71873, #47373 ) ) ;
#47753=ORIENTED_EDGE ( 'NONE', *, *, #109122, .T. ) ;
#47754=EDGE_CURVE ( 'NONE', #103724, #94980, #104396, .T. ) ;
#47755=CIRCLE ( 'NONE', #108383, 0.09999999999999999167 ) ;
#47756=ORIENTED_EDGE ( 'NONE', *, *, #90054, .T. ) ;
#47757=ADVANCED_FACE ( 'NONE', ( #70498 ), #41714, .T. ) ;
#47758=ORIENTED_EDGE ( 'NONE', *, *, #84342, .F. ) ;
#47759=CARTESIAN_POINT ( 'NONE',  ( -6.900000000000019007, 2.500000000000000000, -4.676537180435978769 ) ) ;
#47760=CARTESIAN_POINT ( 'NONE',  ( -13.34999999999999076, 2.500000000000000000, 2.265063509461101354 ) ) ;
#47761=AXIS2_PLACEMENT_3D ( 'NONE', #107297, #49050, #37289 ) ;
#47762=VERTEX_POINT ( 'NONE', #40420 ) ;
#47763=LINE ( 'NONE', #107314, #46443 ) ;
#47764=DIRECTION ( 'NONE',  ( 0.000000000000000000, 0.000000000000000000, 1.000000000000000000 ) ) ;
#47766=DIRECTION ( 'NONE',  ( 0.000000000000000000, 0.000000000000000000, 1.000000000000000000 ) ) ;
#47767=ORIENTED_EDGE ( 'NONE', *, *, #70730, .T. ) ;
#47768=EDGE_CURVE ( 'NONE', #77652, #55549, #12441, .T. ) ;
#47769=CARTESIAN_POINT ( 'NONE',  ( 8.749999999999920064, 2.500000000000000000, -2.857883832488653741 ) ) ;
#47770=CONICAL_SURFACE ( 'NONE', #116702, 0.1000000000000002554, 0.003490658503988666988 ) ;
#47771=DIRECTION ( 'NONE',  ( -0.000000000000000000, -1.000000000000000000, -0.000000000000000000 ) ) ;
#47772=VERTEX_POINT ( 'NONE', #11575 ) ;
#47774=VERTEX_POINT ( 'NONE', #39779 ) ;
#47775=ORIENTED_EDGE ( 'NONE', *, *, #26962, .F. ) ;
#47776=DIRECTION ( 'NONE',  ( 0.000000000000000000, 0.000000000000000000, -1.000000000000000000 ) ) ;
#47777=AXIS2_PLACEMENT_3D ( 'NONE', #126403, #116568, #66816 ) ;
#47778=DIRECTION ( 'NONE',  ( 0.000000000000000000, 0.000000000000000000, 1.000000000000000000 ) ) ;
#47779=EDGE_CURVE ( 'NONE', #60636, #93446, #18708, .T. ) ;
#47780=ORIENTED_EDGE ( 'NONE', *, *, #64013, .F. ) ;
#47781=DIRECTION ( 'NONE',  ( -0.000000000000000000, -1.000000000000000000, -0.000000000000000000 ) ) ;
#47782=DIRECTION ( 'NONE',  ( 0.000000000000000000, 0.000000000000000000, -1.000000000000000000 ) ) ;
#47783=CIRCLE ( 'NONE', #64496, 0.1000000000000002554 ) ;
#47784=DIRECTION ( 'NONE',  ( 0.000000000000000000, 0.000000000000000000, -1.000000000000000000 ) ) ;
#47785=CARTESIAN_POINT ( 'NONE',  ( -1.650000000000034772, 2.500000000000000000, 6.595190528383296780 ) ) ;
#47786=ADVANCED_FACE ( 'NONE', ( #19463 ), #121117, .T. ) ;
#47787=VERTEX_POINT ( 'NONE', #71140 ) ;
#47788=AXIS2_PLACEMENT_3D ( 'NONE', #46273, #16790, #35192 ) ;
#47789=AXIS2_PLACEMENT_3D ( 'NONE', #46320, #86888, #85602 ) ;
#47790=CARTESIAN_POINT ( 'NONE',  ( 10.39999999999991154, 12.50000000000000000, 3.637306695894644726 ) ) ;
#47792=ORIENTED_EDGE ( 'NONE', *, *, #122144, .T. ) ;
#47793=DIRECTION ( 'NONE',  ( 0.000000000000000000, 1.000000000000000000, 0.000000000000000000 ) ) ;
#47794=ADVANCED_FACE ( 'NONE', ( #48943 ), #14481, .T. ) ;
#47795=EDGE_CURVE ( 'NONE', #4367, #65655, #91431, .T. ) ;
#47796=PLANE ( 'NONE',  #87802 ) ;
#47797=ADVANCED_FACE ( 'NONE', ( #88853 ), #21394, .T. ) ;
#47798=FACE_BOUND ( 'NONE', #63568, .T. ) ;
#47799=EDGE_CURVE ( 'NONE', #58927, #22783, #109115, .T. ) ;
#47800=CARTESIAN_POINT ( 'NONE',  ( -5.000000000000022204, 2.500000000000000000, 3.737306695894644371 ) ) ;
#47801=DIRECTION ( 'NONE',  ( 0.000000000000000000, 0.000000000000000000, 1.000000000000000000 ) ) ;
#47802=LINE ( 'NONE', #116523, #119158 ) ;
#47803=EDGE_CURVE ( 'NONE', #46113, #89857, #58437, .T. ) ;
#47804=CIRCLE ( 'NONE', #91614, 0.06509327318403745899 ) ;
#47805=EDGE_LOOP ( 'NONE', ( #18970, #93583 ) ) ;
#47806=CARTESIAN_POINT ( 'NONE',  ( 11.64999999999990443, 2.500000000000000000, -5.702370205355749455 ) ) ;
#47807=DIRECTION ( 'NONE',  ( 0.000000000000000000, 1.000000000000000000, 0.000000000000000000 ) ) ;
#47808=ADVANCED_FACE ( 'NONE', ( #29302 ), #10305, .T. ) ;
#47809=CARTESIAN_POINT ( 'NONE',  ( 3.549999999999943867, 2.500000000000000000, -1.918653347947326004 ) ) ;
#47810=DIRECTION ( 'NONE',  ( -0.000000000000000000, -1.000000000000000000, -0.000000000000000000 ) ) ;
#47811=ORIENTED_EDGE ( 'NONE', *, *, #109535, .T. ) ;
#47812=DIRECTION ( 'NONE',  ( 0.000000000000000000, -0.000000000000000000, 1.000000000000000000 ) ) ;
#47813=EDGE_CURVE ( 'NONE', #94018, #51302, #52164, .T. ) ;
#47814=AXIS2_PLACEMENT_3D ( 'NONE', #128932, #19593, #59552 ) ;
#47815=ADVANCED_FACE ( 'NONE', ( #89501 ), #75150, .T. ) ;
#47816=CONICAL_SURFACE ( 'NONE', #95919, 0.09999999999999982514, 0.003490658503988666988 ) ;
#47817=CARTESIAN_POINT ( 'NONE',  ( -5.850000000000018296, 12.50000000000000000, 7.188010851410848723 ) ) ;
#47818=AXIS2_PLACEMENT_3D ( 'NONE', #100658, #102599, #3763 ) ;
#47819=ORIENTED_EDGE ( 'NONE', *, *, #27649, .T. ) ;
#47820=ORIENTED_EDGE ( 'NONE', *, *, #107023, .F. ) ;
#47821=PLANE ( 'NONE',  #23079 ) ;
#47822=EDGE_CURVE ( 'NONE', #97854, #331, #80973, .T. ) ;
#47823=DIRECTION ( 'NONE',  ( 0.000000000000000000, -0.000000000000000000, 1.000000000000000000 ) ) ;
#47824=FACE_BOUND ( 'NONE', #49176, .T. ) ;
#47825=EDGE_CURVE ( 'NONE', #112012, #9827, #60064, .T. ) ;
#47826=DIRECTION ( 'NONE',  ( -0.000000000000000000, 1.000000000000000000, -0.000000000000000000 ) ) ;
#47827=AXIS2_PLACEMENT_3D ( 'NONE', #127703, #76032, #116589 ) ;
#47828=CIRCLE ( 'NONE', #12298, 0.09999999999999982514 ) ;
#47829=AXIS2_PLACEMENT_3D ( 'NONE', #48867, #128730, #39057 ) ;
#47830=ORIENTED_EDGE ( 'NONE', *, *, #87616, .T. ) ;
#47831=CARTESIAN_POINT ( 'NONE',  ( -1.850000000000033396, 2.500000000000000000, -1.818653347947325916 ) ) ;
#47832=AXIS2_PLACEMENT_3D ( 'NONE', #2110, #40122, #60429 ) ;
#47833=EDGE_LOOP ( 'NONE', ( #22467, #71697 ) ) ;
#47834=ORIENTED_EDGE ( 'NONE', *, *, #122741, .T. ) ;
#47835=CARTESIAN_POINT ( 'NONE',  ( 19.09982477502547127, 0.5559300837585704480, -4.454172625795856710 ) ) ;
#47837=AXIS2_PLACEMENT_3D ( 'NONE', #104459, #34453, #4958 ) ;
#47838=ORIENTED_EDGE ( 'NONE', *, *, #117363, .T. ) ;
#47839=CARTESIAN_POINT ( 'NONE',  ( 5.599999999999931255, 12.50000000000000000, 3.983716857408420076 ) ) ;
#47841=AXIS2_PLACEMENT_3D ( 'NONE', #68674, #127603, #67354 ) ;
#47842=DIRECTION ( 'NONE',  ( 0.000000000000000000, 1.000000000000000000, 0.000000000000000000 ) ) ;
#47843=CARTESIAN_POINT ( 'NONE',  ( 1.649999999999951505, 2.500000000000000000, -2.957883832488653830 ) ) ;
#47844=AXIS2_PLACEMENT_3D ( 'NONE', #121562, #71843, #115438 ) ;
#47845=ORIENTED_EDGE ( 'NONE', *, *, #44116, .F. ) ;
#47846=CARTESIAN_POINT ( 'NONE',  ( 12.69999999999989804, 12.50000000000000000, 0.4115034346978109769 ) ) ;
#47847=CARTESIAN_POINT ( 'NONE',  ( -8.350000000000013856, 2.500000000000000000, -7.288010851410849256 ) ) ;
#47848=DIRECTION ( 'NONE',  ( 0.000000000000000000, 0.000000000000000000, 1.000000000000000000 ) ) ;
#47849=CONICAL_SURFACE ( 'NONE', #120998, 0.1000000000000002554, 0.003490658503988666988 ) ;
#47850=DIRECTION ( 'NONE',  ( -0.000000000000000000, -1.000000000000000000, -0.000000000000000000 ) ) ;
#47851=ORIENTED_EDGE ( 'NONE', *, *, #26220, .T. ) ;
#47852=CARTESIAN_POINT ( 'NONE',  ( -8.750000000000008882, 12.50000000000000000, 1.537336459617582918 ) ) ;
#47853=ORIENTED_EDGE ( 'NONE', *, *, #62722, .F. ) ;
#47854=CARTESIAN_POINT ( 'NONE',  ( 18.00406198521885770, 1.510509990005263647, 4.944015973543540277 ) ) ;
#47855=VERTEX_POINT ( 'NONE', #80333 ) ;
#47856=CARTESIAN_POINT ( 'NONE',  ( -13.54999999999998828, 12.50000000000000000, -2.511473670974875727 ) ) ;
#47857=CARTESIAN_POINT ( 'NONE',  ( 87.50000000000002842, -6.761363245278262823, 3.308765358479927254 ) ) ;
#47859=DIRECTION ( 'NONE',  ( 0.000000000000000000, 1.000000000000000000, 0.000000000000000000 ) ) ;
#47860=CARTESIAN_POINT ( 'NONE',  ( 3.549999999999942091, 2.500000000000000000, 2.511473670974873507 ) ) ;
#47861=EDGE_LOOP ( 'NONE', ( #122122, #63683, #128204, #42326 ) ) ;
#47862=AXIS2_PLACEMENT_3D ( 'NONE', #81549, #31179, #33115 ) ;
#47863=DIRECTION ( 'NONE',  ( -0.000000000000000000, -1.000000000000000000, -0.000000000000000000 ) ) ;
#47864=EDGE_CURVE ( 'NONE', #16549, #60383, #102347, .T. ) ;
#47865=DIRECTION ( 'NONE',  ( 0.000000000000000000, 0.000000000000000000, 1.000000000000000000 ) ) ;
#47866=DIRECTION ( 'NONE',  ( -0.000000000000000000, -1.000000000000000000, -0.000000000000000000 ) ) ;
#47867=DIRECTION ( 'NONE',  ( 0.000000000000000000, 1.000000000000000000, 0.000000000000000000 ) ) ;
#47868=CARTESIAN_POINT ( 'NONE',  ( 8.149999999999923972, 12.50000000000000000, 1.883746621131358934 ) ) ;
#47869=AXIS2_PLACEMENT_3D ( 'NONE', #77872, #108630, #107984 ) ;
#47870=VERTEX_POINT ( 'NONE', #3060 ) ;
#47871=VERTEX_POINT ( 'NONE', #34459 ) ;
#47872=CARTESIAN_POINT ( 'NONE',  ( 1.449999999999950440, 2.500000000000000000, 6.248780366869520542 ) ) ;
#47873=EDGE_LOOP ( 'NONE', ( #73275, #72267, #2507, #61748 ) ) ;
#47874=LINE ( 'NONE', #18395, #103676 ) ;
#47875=VERTEX_POINT ( 'NONE', #114920 ) ;
#47876=ORIENTED_EDGE ( 'NONE', *, *, #65959, .T. ) ;
#47877=ORIENTED_EDGE ( 'NONE', *, *, #76135, .T. ) ;
#47878=CIRCLE ( 'NONE', #123084, 0.1000000000000002554 ) ;
#47879=FACE_OUTER_BOUND ( 'NONE', #61803, .T. ) ;
#47880=CARTESIAN_POINT ( 'NONE',  ( -2.500000000000031086, 12.50000000000000000, 3.637306695894644726 ) ) ;
#47881=CARTESIAN_POINT ( 'NONE',  ( 0.6499999999999543920, 2.500000000000000000, 6.941600689897073018 ) ) ;
#47883=AXIS2_PLACEMENT_3D ( 'NONE', #33961, #45079, #45720 ) ;
#47884=LINE ( 'NONE', #57701, #116224 ) ;
#47885=CARTESIAN_POINT ( 'NONE',  ( 6.649999999999929301, 2.500000000000000000, -2.165063509461101710 ) ) ;
#47887=FACE_OUTER_BOUND ( 'NONE', #38455, .T. ) ;
#47888=CONICAL_SURFACE ( 'NONE', #95992, 0.1000000000000002554, 0.003490658503988666988 ) ;
#47889=VERTEX_POINT ( 'NONE', #73080 ) ;
#47890=PLANE ( 'NONE',  #100051 ) ;
#47891=ORIENTED_EDGE ( 'NONE', *, *, #112731, .T. ) ;
#47892=AXIS2_PLACEMENT_3D ( 'NONE', #122170, #3669, #123436 ) ;
#47893=ORIENTED_EDGE ( 'NONE', *, *, #77237, .T. ) ;
#47894=ORIENTED_EDGE ( 'NONE', *, *, #7111, .F. ) ;
#47895=ORIENTED_EDGE ( 'NONE', *, *, #51067, .F. ) ;
#47896=FACE_OUTER_BOUND ( 'NONE', #30621, .T. ) ;
#47897=ORIENTED_EDGE ( 'NONE', *, *, #69936, .T. ) ;
#47898=ORIENTED_EDGE ( 'NONE', *, *, #93314, .T. ) ;
#47899=EDGE_CURVE ( 'NONE', #121477, #23084, #3690, .T. ) ;
#47901=DIRECTION ( 'NONE',  ( 0.000000000000000000, 1.000000000000000000, 0.000000000000000000 ) ) ;
#47902=CARTESIAN_POINT ( 'NONE',  ( -10.40000000000000213, 2.500000000000000000, 3.637306695894644726 ) ) ;
#47903=CARTESIAN_POINT ( 'NONE',  ( 3.749999999999940492, 2.500000000000000000, 2.857883832488649301 ) ) ;
#47904=CARTESIAN_POINT ( 'NONE',  ( 9.599999999999914380, 2.500000000000000000, 5.022947341949748790 ) ) ;
#47905=CIRCLE ( 'NONE', #75081, 0.1000000000000002554 ) ;
#47906=ORIENTED_EDGE ( 'NONE', *, *, #95780, .T. ) ;
#47907=DIRECTION ( 'NONE',  ( -0.000000000000000000, 1.000000000000000000, -0.000000000000000000 ) ) ;
#47908=ORIENTED_EDGE ( 'NONE', *, *, #45876, .F. ) ;
#47909=AXIS2_PLACEMENT_3D ( 'NONE', #54212, #7013, #16191 ) ;
#47910=DIRECTION ( 'NONE',  ( 0.000000000000000000, 0.000000000000000000, 1.000000000000000000 ) ) ;
#47911=VERTEX_POINT ( 'NONE', #54707 ) ;
#47912=LINE ( 'NONE', #87806, #90150 ) ;
#47913=ORIENTED_EDGE ( 'NONE', *, *, #63752, .F. ) ;
#47914=EDGE_CURVE ( 'NONE', #125307, #21757, #73091, .T. ) ;
#47915=EDGE_CURVE ( 'NONE', #58504, #62036, #4027, .T. ) ;
#47916=EDGE_LOOP ( 'NONE', ( #121133, #83137 ) ) ;
#47917=DIRECTION ( 'NONE',  ( -0.000000000000000000, 1.000000000000000000, -0.000000000000000000 ) ) ;
#47918=CIRCLE ( 'NONE', #112658, 0.1000000000000002554 ) ;
#47919=CARTESIAN_POINT ( 'NONE',  ( 43.29488422903774847, -3.510951914389875750, -3.940494739282157433 ) ) ;
#47920=CIRCLE ( 'NONE', #60542, 0.06509327318403745899 ) ;
#47921=CIRCLE ( 'NONE', #87603, 0.06509327318403745899 ) ;
#47922=DIRECTION ( 'NONE',  ( 0.000000000000000000, 1.000000000000000000, 0.000000000000000000 ) ) ;
#47923=FACE_OUTER_BOUND ( 'NONE', #105607, .T. ) ;
#47924=DIRECTION ( 'NONE',  ( -4.274815082592931898E-19, -0.9999939076577903929, -0.003490651415223739937 ) ) ;
#47925=ORIENTED_EDGE ( 'NONE', *, *, #95412, .F. ) ;
#47926=DIRECTION ( 'NONE',  ( 0.000000000000000000, 0.000000000000000000, 1.000000000000000000 ) ) ;
#47927=DIRECTION ( 'NONE',  ( 0.000000000000000000, -0.9999939076577903929, 0.003490651415223739937 ) ) ;
#47928=EDGE_CURVE ( 'NONE', #48277, #90721, #77209, .T. ) ;
#47929=CARTESIAN_POINT ( 'NONE',  ( -3.150000000000030553, 2.500000000000000000, 6.148780366869520009 ) ) ;
#47930=CARTESIAN_POINT ( 'NONE',  ( -12.29999999999999538, 12.50000000000000000, -0.3464101615137741841 ) ) ;
#47931=AXIS2_PLACEMENT_3D ( 'NONE', #12685, #119421, #91914 ) ;
#47932=CARTESIAN_POINT ( 'NONE',  ( 7.499999999999927169, 2.500000000000000000, 3.637306695894644726 ) ) ;
#47933=AXIS2_PLACEMENT_3D ( 'NONE', #97180, #124229, #38270 ) ;
#47934=EDGE_LOOP ( 'NONE', ( #67495, #123541, #27488, #93535 ) ) ;
#47935=ORIENTED_EDGE ( 'NONE', *, *, #96812, .F. ) ;
#47936=LINE ( 'NONE', #108761, #123993 ) ;
#47938=CARTESIAN_POINT ( 'NONE',  ( 14.19999999999989626, 2.500000000000000000, -2.276824562219559311E-15 ) ) ;
#47939=DIRECTION ( 'NONE',  ( 0.000000000000000000, 1.000000000000000000, 0.000000000000000000 ) ) ;
#47940=VERTEX_POINT ( 'NONE', #113003 ) ;
#47942=DIRECTION ( 'NONE',  ( -0.000000000000000000, -1.000000000000000000, -0.000000000000000000 ) ) ;
#47943=FACE_OUTER_BOUND ( 'NONE', #116673, .T. ) ;
#47944=DIRECTION ( 'NONE',  ( 0.000000000000000000, 1.000000000000000000, 0.000000000000000000 ) ) ;
#47945=ORIENTED_EDGE ( 'NONE', *, *, #5098, .T. ) ;
#47946=EDGE_CURVE ( 'NONE', #100782, #122978, #2377, .T. ) ;
#47947=DIRECTION ( 'NONE',  ( 0.000000000000000000, 1.000000000000000000, 0.000000000000000000 ) ) ;
#47948=DIRECTION ( 'NONE',  ( -0.000000000000000000, -1.000000000000000000, -0.000000000000000000 ) ) ;
#47949=EDGE_LOOP ( 'NONE', ( #39460, #36873, #26573, #31837 ) ) ;
#47950=ADVANCED_FACE ( 'NONE', ( #25245 ), #98211, .T. ) ;
#47951=LINE ( 'NONE', #55190, #107067 ) ;
#47952=CIRCLE ( 'NONE', #77195, 0.1000000000000000056 ) ;
#47953=DIRECTION ( 'NONE',  ( 0.000000000000000000, 0.000000000000000000, 1.000000000000000000 ) ) ;
#47954=ADVANCED_FACE ( 'NONE', ( #82910 ), #52155, .T. ) ;
#47955=CARTESIAN_POINT ( 'NONE',  ( 11.89999999999990798, 12.50000000000000000, 3.918623584224383727 ) ) ;
#47957=DIRECTION ( 'NONE',  ( -0.000000000000000000, -1.000000000000000000, -0.000000000000000000 ) ) ;
#47958=ADVANCED_FACE ( 'NONE', ( #103185 ), #16715, .T. ) ;
#47959=EDGE_CURVE ( 'NONE', #111595, #17095, #119148, .T. ) ;
#47960=ORIENTED_EDGE ( 'NONE', *, *, #112377, .F. ) ;
#47961=CARTESIAN_POINT ( 'NONE',  ( -8.950000000000008171, 2.500000000000000000, 1.718653347947321386 ) ) ;
#47962=AXIS2_PLACEMENT_3D ( 'NONE', #101644, #14359, #32280 ) ;
#47963=CARTESIAN_POINT ( 'NONE',  ( 11.64999999999990443, 12.50000000000000000, 1.472243186433545459 ) ) ;
#47964=EDGE_CURVE ( 'NONE', #42047, #126587, #13499, .T. ) ;
#47965=EDGE_CURVE ( 'NONE', #39568, #8482, #14582, .T. ) ;
#47966=CARTESIAN_POINT ( 'NONE',  ( -1.850000000000033396, 2.500000000000000000, -2.611473670974877592 ) ) ;
#47967=ORIENTED_EDGE ( 'NONE', *, *, #1907, .F. ) ;
#47968=DIRECTION ( 'NONE',  ( -0.000000000000000000, 1.000000000000000000, -0.000000000000000000 ) ) ;
#47969=AXIS2_PLACEMENT_3D ( 'NONE', #111001, #32495, #20718 ) ;
#47970=AXIS2_PLACEMENT_3D ( 'NONE', #51517, #29943, #69197 ) ;
#47971=EDGE_CURVE ( 'NONE', #4778, #90560, #123268, .T. ) ;
#47972=CARTESIAN_POINT ( 'NONE',  ( -6.450000000000016165, 12.50000000000000000, 2.446380397790835826 ) ) ;
#47973=CIRCLE ( 'NONE', #45913, 0.06509327318403741736 ) ;
#47974=ORIENTED_EDGE ( 'NONE', *, *, #69500, .F. ) ;
#47975=DIRECTION ( 'NONE',  ( 0.000000000000000000, 0.000000000000000000, 1.000000000000000000 ) ) ;
#47976=ORIENTED_EDGE ( 'NONE', *, *, #41304, .T. ) ;
#47977=ADVANCED_FACE ( 'NONE', ( #23987 ), #66807, .T. ) ;
#47978=CARTESIAN_POINT ( 'NONE',  ( 9.199999999999919353, 12.50000000000000000, -2.276824562219559311E-15 ) ) ;
#47979=CONICAL_SURFACE ( 'NONE', #70954, 0.09999999999999999167, 0.003490658503988666988 ) ;
#47980=CIRCLE ( 'NONE', #64686, 0.06509327318403745899 ) ;
#47981=VERTEX_POINT ( 'NONE', #122190 ) ;
#47982=DIRECTION ( 'NONE',  ( 0.000000000000000000, 1.000000000000000000, 0.000000000000000000 ) ) ;
#47983=FACE_OUTER_BOUND ( 'NONE', #115851, .T. ) ;
#47984=ORIENTED_EDGE ( 'NONE', *, *, #26004, .F. ) ;
#47985=ORIENTED_EDGE ( 'NONE', *, *, #27051, .T. ) ;
#47986=CARTESIAN_POINT ( 'NONE',  ( -4.800000000000024691, 12.50000000000000000, 0.2813168883297361700 ) ) ;
#47987=DIRECTION ( 'NONE',  ( -4.274815082592931898E-19, -0.9999939076577903929, -0.003490651415223739937 ) ) ;
#47988=VERTEX_POINT ( 'NONE', #44250 ) ;
#47989=CARTESIAN_POINT ( 'NONE',  ( -10.60000000000000320, 12.50000000000000000, -4.741630453620010677 ) ) ;
#47990=DIRECTION ( 'NONE',  ( 0.000000000000000000, 1.000000000000000000, 0.000000000000000000 ) ) ;
#47991=DIRECTION ( 'NONE',  ( 0.000000000000000000, 1.000000000000000000, 0.000000000000000000 ) ) ;
#47992=CONICAL_SURFACE ( 'NONE', #52105, 0.1000000000000002554, 0.003490658503988666988 ) ;
#47993=DIRECTION ( 'NONE',  ( 0.000000000000000000, -0.9999939076577903929, 0.003490651415223739937 ) ) ;
#47994=DIRECTION ( 'NONE',  ( 0.000000000000000000, 0.000000000000000000, 1.000000000000000000 ) ) ;
#47995=DIRECTION ( 'NONE',  ( -0.000000000000000000, -1.000000000000000000, -0.000000000000000000 ) ) ;
#47996=VECTOR ( 'NONE', #99132, 1000.000000000000000 ) ;
#47997=CONICAL_SURFACE ( 'NONE', #64704, 0.1000000000000002554, 0.003490658503988666988 ) ;
#47998=VERTEX_POINT ( 'NONE', #84823 ) ;
#47999=ORIENTED_EDGE ( 'NONE', *, *, #19285, .F. ) ;
#48000=ORIENTED_EDGE ( 'NONE', *, *, #34382, .T. ) ;
#48001=VERTEX_POINT ( 'NONE', #65164 ) ;
#48002=CARTESIAN_POINT ( 'NONE',  ( 2.099999999999949463, 2.500000000000000000, -3.737306695894649700 ) ) ;
#48003=LINE ( 'NONE', #115405, #44887 ) ;
#48004=DIRECTION ( 'NONE',  ( -0.000000000000000000, 1.000000000000000000, -0.000000000000000000 ) ) ;
#48005=ORIENTED_EDGE ( 'NONE', *, *, #13351, .T. ) ;
#48006=FACE_BOUND ( 'NONE', #84582, .T. ) ;
#48007=ORIENTED_EDGE ( 'NONE', *, *, #9839, .F. ) ;
#48008=DIRECTION ( 'NONE',  ( -0.000000000000000000, 1.000000000000000000, -0.000000000000000000 ) ) ;
#48009=DIRECTION ( 'NONE',  ( -4.274815082592931898E-19, -0.9999939076577903929, -0.003490651415223739937 ) ) ;
#48010=AXIS2_PLACEMENT_3D ( 'NONE', #3621, #43567, #123388 ) ;
#48011=CONICAL_SURFACE ( 'NONE', #129592, 0.09999999999999982514, 0.003490658503988666988 ) ;
#48012=CARTESIAN_POINT ( 'NONE',  ( -13.54999999999998828, 2.500000000000000000, 1.818653347947325472 ) ) ;
#48013=CIRCLE ( 'NONE', #121156, 0.09999999999999999167 ) ;
#48014=EDGE_CURVE ( 'NONE', #24036, #98383, #33491, .T. ) ;
#48015=CARTESIAN_POINT ( 'NONE',  ( 14.54999999999989235, 2.500000000000000000, -2.065063509461102065 ) ) ;
#48016=DIRECTION ( 'NONE',  ( 0.000000000000000000, 1.000000000000000000, 0.000000000000000000 ) ) ;
#48017=LINE ( 'NONE', #16586, #41251 ) ;
#48018=CARTESIAN_POINT ( 'NONE',  ( -12.09999999999999609, 12.50000000000000000, -4.330127018922198978 ) ) ;
#48019=PLANE ( 'NONE',  #93115 ) ;
#48020=DIRECTION ( 'NONE',  ( 0.000000000000000000, 0.000000000000000000, -1.000000000000000000 ) ) ;
#48021=CIRCLE ( 'NONE', #12494, 0.06509327318403745899 ) ;
#48022=FACE_OUTER_BOUND ( 'NONE', #44531, .T. ) ;
#48023=EDGE_CURVE ( 'NONE', #32647, #92549, #43868, .T. ) ;
#48024=AXIS2_PLACEMENT_3D ( 'NONE', #120050, #59210, #110851 ) ;
#48025=ORIENTED_EDGE ( 'NONE', *, *, #100556, .F. ) ;
#48026=ORIENTED_EDGE ( 'NONE', *, *, #66211, .F. ) ;
#48027=VECTOR ( 'NONE', #128466, 1000.000000000000000 ) ;
#48028=EDGE_LOOP ( 'NONE', ( #8412, #101481 ) ) ;
#48029=ORIENTED_EDGE ( 'NONE', *, *, #124328, .F. ) ;
#48030=CARTESIAN_POINT ( 'NONE',  ( 16.55874544816221317, -0.4845305829210151960, -6.091953208799018249 ) ) ;
#48031=CARTESIAN_POINT ( 'NONE',  ( -2.100000000000033396, 2.500000000000000000, -5.022947341949754119 ) ) ;
#48032=EDGE_LOOP ( 'NONE', ( #89799, #47380 ) ) ;
#48033=ORIENTED_EDGE ( 'NONE', *, *, #121232, .F. ) ;
#48034=EDGE_LOOP ( 'NONE', ( #28247, #11136, #115320, #76080 ) ) ;
#48035=DIRECTION ( 'NONE',  ( 0.000000000000000000, 0.000000000000000000, 1.000000000000000000 ) ) ;
#48036=LINE ( 'NONE', #77478, #66436 ) ;
#48037=CARTESIAN_POINT ( 'NONE',  ( -5.200000000000022382, 12.50000000000000000, 0.3464101615137735735 ) ) ;
#48038=CARTESIAN_POINT ( 'NONE',  ( 0.8499999999999536815, 2.500000000000000000, 5.902370205355745192 ) ) ;
#48040=CARTESIAN_POINT ( 'NONE',  ( 0.5999999999999551248, 12.50000000000000000, -4.741630453620016006 ) ) ;
#48041=DIRECTION ( 'NONE',  ( 0.000000000000000000, 0.000000000000000000, 1.000000000000000000 ) ) ;
#48042=ORIENTED_EDGE ( 'NONE', *, *, #41010, .T. ) ;
#48043=PLANE ( 'NONE',  #60170 ) ;
#48044=ORIENTED_EDGE ( 'NONE', *, *, #13774, .T. ) ;
#48045=EDGE_LOOP ( 'NONE', ( #34479, #8207 ) ) ;
#48046=ORIENTED_EDGE ( 'NONE', *, *, #75683, .T. ) ;
#48047=DIRECTION ( 'NONE',  ( -0.000000000000000000, -1.000000000000000000, -0.000000000000000000 ) ) ;
#48048=ORIENTED_EDGE ( 'NONE', *, *, #108666, .T. ) ;
#48049=ORIENTED_EDGE ( 'NONE', *, *, #104781, .F. ) ;
#48050=CARTESIAN_POINT ( 'NONE',  ( 5.599999999999931255, 2.500000000000000000, 3.883716857408420431 ) ) ;
#48051=ADVANCED_FACE ( 'NONE', ( #126029 ), #37601, .T. ) ;
#48052=CARTESIAN_POINT ( 'NONE',  ( -12.04999999999999716, 2.500000000000000000, -6.495190528383298911 ) ) ;
#48053=CARTESIAN_POINT ( 'NONE',  ( 10.84999999999990905, 2.500000000000000000, 2.857883832488649301 ) ) ;
#48054=DIRECTION ( 'NONE',  ( 0.000000000000000000, 1.000000000000000000, 0.000000000000000000 ) ) ;
#48055=DIRECTION ( 'NONE',  ( -4.274815082592931898E-19, -0.9999939076577903929, -0.003490651415223739937 ) ) ;
#48056=CIRCLE ( 'NONE', #116976, 0.09999999999999982514 ) ;
#48057=ORIENTED_EDGE ( 'NONE', *, *, #23445, .T. ) ;
#48058=DIRECTION ( 'NONE',  ( -0.000000000000000000, -1.000000000000000000, -0.000000000000000000 ) ) ;
#48059=ADVANCED_FACE ( 'NONE', ( #126698 ), #87740, .T. ) ;
#48060=VERTEX_POINT ( 'NONE', #38320 ) ;
#48061=DIRECTION ( 'NONE',  ( 0.000000000000000000, 1.000000000000000000, 0.000000000000000000 ) ) ;
#48062=CIRCLE ( 'NONE', #11, 0.09999999999999982514 ) ;
#48063=AXIS2_PLACEMENT_3D ( 'NONE', #44917, #53453, #112369 ) ;
#48066=CARTESIAN_POINT ( 'NONE',  ( 5.399999999999936406, 2.500000000000000000, -3.637306695894650055 ) ) ;
#48067=VERTEX_POINT ( 'NONE', #35734 ) ;
#48068=CARTESIAN_POINT ( 'NONE',  ( 4.349999999999937472, 2.500000000000000000, 6.941600689897073018 ) ) ;
#48069=EDGE_CURVE ( 'NONE', #35458, #38872, #95300, .T. ) ;
#48070=CARTESIAN_POINT ( 'NONE',  ( 10.44999999999991047, 12.50000000000000000, -6.495190528383302464 ) ) ;
#48071=ADVANCED_FACE ( 'NONE', ( #95941 ), #100284, .T. ) ;
#48072=VERTEX_POINT ( 'NONE', #78250 ) ;
#48073=AXIS2_PLACEMENT_3D ( 'NONE', #55165, #26996, #125812 ) ;
#48074=AXIS2_PLACEMENT_3D ( 'NONE', #117148, #67396, #127639 ) ;
#48075=ADVANCED_FACE ( 'NONE', ( #37027 ), #114931, .T. ) ;
#48076=CARTESIAN_POINT ( 'NONE',  ( 1.249999999999952038, 12.50000000000000000, -1.537336459617587581 ) ) ;
#48077=ORIENTED_EDGE ( 'NONE', *, *, #76204, .F. ) ;
#48078=EDGE_LOOP ( 'NONE', ( #55559, #107209, #104417, #31414 ) ) ;
#48079=CARTESIAN_POINT ( 'NONE',  ( 97.50000000000000000, 0.000000000000000000, 0.000000000000000000 ) ) ;
#48080=DIRECTION ( 'NONE',  ( -0.000000000000000000, -1.000000000000000000, -0.000000000000000000 ) ) ;
#48081=ADVANCED_FACE ( 'NONE', ( #17354 ), #76950, .T. ) ;
#48083=DIRECTION ( 'NONE',  ( 0.000000000000000000, 0.000000000000000000, 1.000000000000000000 ) ) ;
#48084=DIRECTION ( 'NONE',  ( 0.000000000000000000, 0.000000000000000000, 1.000000000000000000 ) ) ;
#48085=CARTESIAN_POINT ( 'NONE',  ( 5.849999999999933031, 2.500000000000000000, 7.188010851410848723 ) ) ;
#48086=VERTEX_POINT ( 'NONE', #76306 ) ;
#48087=DIRECTION ( 'NONE',  ( 0.000000000000000000, 0.000000000000000000, 1.000000000000000000 ) ) ;
#48088=CARTESIAN_POINT ( 'NONE',  ( -3.350000000000028955, 2.500000000000000000, 7.288010851410849256 ) ) ;
#48089=VECTOR ( 'NONE', #46720, 1000.000000000000000 ) ;
#48090=ORIENTED_EDGE ( 'NONE', *, *, #109409, .F. ) ;
#48091=DIRECTION ( 'NONE',  ( 0.000000000000000000, 1.000000000000000000, 0.000000000000000000 ) ) ;
#48092=CARTESIAN_POINT ( 'NONE',  ( -9.400000000000007461, 12.50000000000000000, 0.3464101615137735735 ) ) ;
#48093=DIRECTION ( 'NONE',  ( 0.000000000000000000, 0.000000000000000000, 1.000000000000000000 ) ) ;
#48094=CARTESIAN_POINT ( 'NONE',  ( 11.64999999999990798, 12.50000000000000000, 5.802370205355744659 ) ) ;
#48096=ORIENTED_EDGE ( 'NONE', *, *, #51806, .F. ) ;
#48097=AXIS2_PLACEMENT_3D ( 'NONE', #115703, #65969, #26053 ) ;
#48098=CARTESIAN_POINT ( 'NONE',  ( 9.349999999999916156, 2.500000000000000000, -1.818653347947326138 ) ) ;
#48099=CARTESIAN_POINT ( 'NONE',  ( 14.54999999999989235, 2.500000000000000000, -2.065063509461102065 ) ) ;
#48100=CIRCLE ( 'NONE', #121260, 0.06509327318403745899 ) ;
#48101=VERTEX_POINT ( 'NONE', #118153 ) ;
#48102=EDGE_CURVE ( 'NONE', #28983, #97899, #56447, .T. ) ;
#48103=FACE_OUTER_BOUND ( 'NONE', #32527, .T. ) ;
#48104=CIRCLE ( 'NONE', #2119, 0.06509327318403745899 ) ;
#48105=AXIS2_PLACEMENT_3D ( 'NONE', #37346, #58910, #8495 ) ;
#48106=VERTEX_POINT ( 'NONE', #87393 ) ;
#48107=ORIENTED_EDGE ( 'NONE', *, *, #78409, .T. ) ;
#48108=CARTESIAN_POINT ( 'NONE',  ( -12.09999999999999609, 12.50000000000000000, -0.6277270498435126855 ) ) ;
#48109=EDGE_CURVE ( 'NONE', #13047, #39415, #4117, .T. ) ;
#48111=VERTEX_POINT ( 'NONE', #127347 ) ;
#48112=DIRECTION ( 'NONE',  ( 0.000000000000000000, 0.000000000000000000, 1.000000000000000000 ) ) ;
#48113=CARTESIAN_POINT ( 'NONE',  ( -2.900000000000030553, 12.50000000000000000, 5.022947341949748790 ) ) ;
#48114=EDGE_CURVE ( 'NONE', #64820, #24778, #105101, .T. ) ;
#48115=CIRCLE ( 'NONE', #123323, 0.06509327318403745899 ) ;
#48116=EDGE_CURVE ( 'NONE', #12607, #117167, #85697, .T. ) ;
#48117=CARTESIAN_POINT ( 'NONE',  ( -2.100000000000033396, 2.500000000000000000, -4.922947341949753586 ) ) ;
#48118=ORIENTED_EDGE ( 'NONE', *, *, #109246, .F. ) ;
#48119=PLANE ( 'NONE',  #25755 ) ;
#48120=ADVANCED_FACE ( 'NONE', ( #16066 ), #104475, .T. ) ;
#48121=CARTESIAN_POINT ( 'NONE',  ( 9.799999999999915445, 12.50000000000000000, 3.983716857408420964 ) ) ;
#48122=ORIENTED_EDGE ( 'NONE', *, *, #119423, .F. ) ;
#48123=CARTESIAN_POINT ( 'NONE',  ( -9.350000000000006750, 12.50000000000000000, -1.818653347947325916 ) ) ;
#48124=CARTESIAN_POINT ( 'NONE',  ( -10.80000000000000249, 12.50000000000000000, -4.265033745738159965 ) ) ;
#48125=ORIENTED_EDGE ( 'NONE', *, *, #127445, .F. ) ;
#48126=ADVANCED_FACE ( 'NONE', ( #127973 ), #7544, .T. ) ;
#48127=EDGE_CURVE ( 'NONE', #110840, #58034, #94014, .T. ) ;
#48128=VERTEX_POINT ( 'NONE', #16707 ) ;
#48129=ORIENTED_EDGE ( 'NONE', *, *, #25479, .T. ) ;
#48130=CARTESIAN_POINT ( 'NONE',  ( -5.450000000000023270, 12.50000000000000000, -2.099970236277064473 ) ) ;
#48131=DIRECTION ( 'NONE',  ( 0.000000000000000000, 0.000000000000000000, 1.000000000000000000 ) ) ;
#48132=DIRECTION ( 'NONE',  ( -4.274815082592931898E-19, -0.9999939076577903929, -0.003490651415223739937 ) ) ;
#48133=FACE_BOUND ( 'NONE', #23581, .T. ) ;
#48134=EDGE_LOOP ( 'NONE', ( #22292, #85405, #100527, #17175 ) ) ;
#48135=FACE_OUTER_BOUND ( 'NONE', #59929, .T. ) ;
#48136=DIRECTION ( 'NONE',  ( -0.000000000000000000, -1.000000000000000000, -0.000000000000000000 ) ) ;
#48137=EDGE_LOOP ( 'NONE', ( #38813, #97530 ) ) ;
#48138=CARTESIAN_POINT ( 'NONE',  ( -11.64999999999999858, 2.500000000000000000, -5.802370205355746435 ) ) ;
#48139=CARTESIAN_POINT ( 'NONE',  ( 17.49862860983209956, 2.500000000000000000, 4.081131818001135336 ) ) ;
#48140=AXIS2_PLACEMENT_3D ( 'NONE', #26478, #4233, #104386 ) ;
#48141=CARTESIAN_POINT ( 'NONE',  ( 11.84999999999990727, 12.50000000000000000, 6.906693963081109722 ) ) ;
#48142=DIRECTION ( 'NONE',  ( -0.000000000000000000, -1.000000000000000000, -0.000000000000000000 ) ) ;
#48143=AXIS2_PLACEMENT_3D ( 'NONE', #105826, #15499, #24696 ) ;
#48144=PLANE ( 'NONE',  #1250 ) ;
#48145=LINE ( 'NONE', #40927, #2307 ) ;
#48146=VECTOR ( 'NONE', #123274, 1000.000000000000000 ) ;
#48147=AXIS2_PLACEMENT_3D ( 'NONE', #122031, #32388, #72293 ) ;
#48148=ORIENTED_EDGE ( 'NONE', *, *, #75758, .T. ) ;
#48149=ORIENTED_EDGE ( 'NONE', *, *, #71309, .T. ) ;
#48150=ORIENTED_EDGE ( 'NONE', *, *, #55734, .T. ) ;
#48151=ORIENTED_EDGE ( 'NONE', *, *, #123783, .F. ) ;
#48152=ORIENTED_EDGE ( 'NONE', *, *, #118434, .T. ) ;
#48153=LINE ( 'NONE', #78916, #111195 ) ;
#48154=DIRECTION ( 'NONE',  ( 0.000000000000000000, -0.000000000000000000, 1.000000000000000000 ) ) ;
#48155=ORIENTED_EDGE ( 'NONE', *, *, #123324, .T. ) ;
#48156=FACE_BOUND ( 'NONE', #30535, .T. ) ;
#48157=DIRECTION ( 'NONE',  ( 0.000000000000000000, 0.000000000000000000, 1.000000000000000000 ) ) ;
#48158=CARTESIAN_POINT ( 'NONE',  ( 11.24999999999990941, 2.500000000000000000, -1.372243186433550033 ) ) ;
#48159=DIRECTION ( 'NONE',  ( -0.000000000000000000, 1.000000000000000000, -0.000000000000000000 ) ) ;
#48160=DIRECTION ( 'NONE',  ( 0.000000000000000000, 0.000000000000000000, -1.000000000000000000 ) ) ;
#48161=CARTESIAN_POINT ( 'NONE',  ( 5.849999999999931255, 12.50000000000000000, 2.857883832488649301 ) ) ;
#48162=ORIENTED_EDGE ( 'NONE', *, *, #92999, .F. ) ;
#48163=DIRECTION ( 'NONE',  ( 0.000000000000000000, 0.000000000000000000, -1.000000000000000000 ) ) ;
#48165=EDGE_CURVE ( 'NONE', #2125, #104031, #91967, .T. ) ;
#48166=ORIENTED_EDGE ( 'NONE', *, *, #19461, .T. ) ;
#48167=VERTEX_POINT ( 'NONE', #29774 ) ;
#48168=CARTESIAN_POINT ( 'NONE',  ( -4.350000000000023626, 12.50000000000000000, -1.818653347947325916 ) ) ;
#48169=CARTESIAN_POINT ( 'NONE',  ( -8.100000000000010303, 12.50000000000000000, 4.741630453620009789 ) ) ;
#48170=FACE_OUTER_BOUND ( 'NONE', #89866, .T. ) ;
#48171=ORIENTED_EDGE ( 'NONE', *, *, #97617, .T. ) ;
#48172=DIRECTION ( 'NONE',  ( 0.000000000000000000, 0.000000000000000000, 1.000000000000000000 ) ) ;
#48173=VECTOR ( 'NONE', #122422, 1000.000000000000000 ) ;
#48174=CARTESIAN_POINT ( 'NONE',  ( 1.049999999999954081, 12.50000000000000000, -6.148780366869526226 ) ) ;
#48175=AXIS2_PLACEMENT_3D ( 'NONE', #73791, #32623, #92143 ) ;
#48176=LINE ( 'NONE', #59307, #123034 ) ;
#48178=DIRECTION ( 'NONE',  ( 0.000000000000000000, 0.000000000000000000, 1.000000000000000000 ) ) ;
#48179=DIRECTION ( 'NONE',  ( 0.000000000000000000, 1.000000000000000000, 0.000000000000000000 ) ) ;
#48180=DIRECTION ( 'NONE',  ( -0.000000000000000000, -1.000000000000000000, -0.000000000000000000 ) ) ;
#48181=ORIENTED_EDGE ( 'NONE', *, *, #82389, .T. ) ;
#48182=CARTESIAN_POINT ( 'NONE',  ( -7.500000000000015099, 12.50000000000000000, -0.7579135962115916003 ) ) ;
#48183=AXIS2_PLACEMENT_3D ( 'NONE', #99305, #20739, #70479 ) ;
#48184=ORIENTED_EDGE ( 'NONE', *, *, #77817, .T. ) ;
#48185=ORIENTED_EDGE ( 'NONE', *, *, #105000, .T. ) ;
#48186=DIRECTION ( 'NONE',  ( 0.000000000000000000, 0.000000000000000000, -1.000000000000000000 ) ) ;
#48187=CARTESIAN_POINT ( 'NONE',  ( 4.999999999999936939, 12.50000000000000000, -0.6928203230275541413 ) ) ;
#48188=DIRECTION ( 'NONE',  ( -0.000000000000000000, 1.000000000000000000, -0.000000000000000000 ) ) ;
#48189=ORIENTED_EDGE ( 'NONE', *, *, #35542, .T. ) ;
#48190=ORIENTED_EDGE ( 'NONE', *, *, #123460, .F. ) ;
#48191=CONICAL_SURFACE ( 'NONE', #121342, 0.1000000000000000056, 0.003490658503988666988 ) ;
#48192=DIRECTION ( 'NONE',  ( 0.000000000000000000, 1.000000000000000000, 0.000000000000000000 ) ) ;
#48193=AXIS2_PLACEMENT_3D ( 'NONE', #35883, #75791, #126193 ) ;
#48194=LINE ( 'NONE', #88767, #116358 ) ;
#48195=DIRECTION ( 'NONE',  ( 0.000000000000000000, 0.000000000000000000, 1.000000000000000000 ) ) ;
#48196=ORIENTED_EDGE ( 'NONE', *, *, #127729, .F. ) ;
#48197=ORIENTED_EDGE ( 'NONE', *, *, #215, .F. ) ;
#48198=DIRECTION ( 'NONE',  ( 0.000000000000000000, 0.000000000000000000, 1.000000000000000000 ) ) ;
#48199=CIRCLE ( 'NONE', #44013, 0.09999999999999982514 ) ;
#48200=EDGE_LOOP ( 'NONE', ( #100185, #42595, #45490, #37500 ) ) ;
#48201=CARTESIAN_POINT ( 'NONE',  ( 11.04999999999990834, 2.500000000000000000, 1.918653347947321564 ) ) ;
#48202=ADVANCED_FACE ( 'NONE', ( #91274 ), #64767, .T. ) ;
#48203=DIRECTION ( 'NONE',  ( 0.000000000000000000, -0.9999939076577903929, 0.003490651415223739937 ) ) ;
#48204=VERTEX_POINT ( 'NONE', #50701 ) ;
#48205=CARTESIAN_POINT ( 'NONE',  ( 8.749999999999953815, 12.50000000000000000, 6.495190528383297135 ) ) ;
#48206=CARTESIAN_POINT ( 'NONE',  ( 7.049999999999928768, 2.500000000000000000, 6.495190528383297135 ) ) ;
#48207=VECTOR ( 'NONE', #108338, 1000.000000000000000 ) ;
#48208=CARTESIAN_POINT ( 'NONE',  ( -7.499999999999980460, 2.500000000000000000, -4.230127018922201998 ) ) ;
#48209=EDGE_CURVE ( 'NONE', #87979, #26681, #121202, .T. ) ;
#48210=DIRECTION ( 'NONE',  ( 0.000000000000000000, 0.000000000000000000, 1.000000000000000000 ) ) ;
#48211=EDGE_CURVE ( 'NONE', #51042, #27361, #108681, .T. ) ;
#48212=ORIENTED_EDGE ( 'NONE', *, *, #52723, .F. ) ;
#48213=CARTESIAN_POINT ( 'NONE',  ( -2.700000000000029932, 2.500000000000000000, -0.4464101615137782142 ) ) ;
#48214=ADVANCED_FACE ( 'NONE', ( #41551 ), #46007, .T. ) ;
#48215=ORIENTED_EDGE ( 'NONE', *, *, #81648, .F. ) ;
#48216=EDGE_CURVE ( 'NONE', #44822, #80384, #18666, .T. ) ;
#48217=ORIENTED_EDGE ( 'NONE', *, *, #53399, .F. ) ;
#48218=EDGE_CURVE ( 'NONE', #74651, #48167, #110269, .T. ) ;
#48219=DIRECTION ( 'NONE',  ( 0.000000000000000000, 1.000000000000000000, 0.000000000000000000 ) ) ;
#48221=DIRECTION ( 'NONE',  ( 0.000000000000000000, 0.000000000000000000, -1.000000000000000000 ) ) ;
#48222=EDGE_CURVE ( 'NONE', #102784, #25279, #10474, .T. ) ;
#48223=DIRECTION ( 'NONE',  ( 0.000000000000000000, 0.000000000000000000, 1.000000000000000000 ) ) ;
#48224=DIRECTION ( 'NONE',  ( -0.000000000000000000, -1.000000000000000000, -0.000000000000000000 ) ) ;
#48225=CARTESIAN_POINT ( 'NONE',  ( -10.65000000000000391, 12.50000000000000000, -6.841600689897075149 ) ) ;
#48226=DIRECTION ( 'NONE',  ( 0.000000000000000000, 0.000000000000000000, -1.000000000000000000 ) ) ;
#48227=CARTESIAN_POINT ( 'NONE',  ( -1.650000000000034772, 2.500000000000000000, 1.572243186433545548 ) ) ;
#48228=CARTESIAN_POINT ( 'NONE',  ( -6.650000000000019007, 2.500000000000000000, -1.372243186433550033 ) ) ;
#48229=AXIS2_PLACEMENT_3D ( 'NONE', #84089, #86010, #124021 ) ;
#48230=CIRCLE ( 'NONE', #52427, 0.09999999999999982514 ) ;
#48231=AXIS2_PLACEMENT_3D ( 'NONE', #33094, #23236, #110339 ) ;
#48232=EDGE_CURVE ( 'NONE', #61265, #3657, #78897, .T. ) ;
#48233=FACE_OUTER_BOUND ( 'NONE', #48587, .T. ) ;
#48234=AXIS2_PLACEMENT_3D ( 'NONE', #59714, #29577, #119246 ) ;
#48235=EDGE_LOOP ( 'NONE', ( #21375, #58500, #69522, #71074 ) ) ;
#48236=CARTESIAN_POINT ( 'NONE',  ( 13.94999999999989448, 2.500000000000000000, -2.511473670974877948 ) ) ;
#48237=CIRCLE ( 'NONE', #121391, 0.06509327318403745899 ) ;
#48238=LINE ( 'NONE', #109060, #20741 ) ;
#48240=CARTESIAN_POINT ( 'NONE',  ( 2.099999999999950351, 12.50000000000000000, -0.6928203230275541413 ) ) ;
#48241=DIRECTION ( 'NONE',  ( 0.000000000000000000, -0.9999939076577903929, 0.003490651415223739937 ) ) ;
#48242=ORIENTED_EDGE ( 'NONE', *, *, #25418, .F. ) ;
#48243=DIRECTION ( 'NONE',  ( 0.000000000000000000, 0.000000000000000000, 1.000000000000000000 ) ) ;
#48245=CARTESIAN_POINT ( 'NONE',  ( -6.850000000000013856, 2.500000000000000000, 1.718653347947321386 ) ) ;
#48246=EDGE_LOOP ( 'NONE', ( #21215, #67121, #101889, #93969 ) ) ;
#48247=EDGE_LOOP ( 'NONE', ( #8171, #96298 ) ) ;
#48248=FACE_OUTER_BOUND ( 'NONE', #12102, .T. ) ;
#48249=EDGE_LOOP ( 'NONE', ( #40845, #42273 ) ) ;
#48250=ORIENTED_EDGE ( 'NONE', *, *, #55020, .T. ) ;
#48251=EDGE_LOOP ( 'NONE', ( #69029, #75652, #20698, #117940 ) ) ;
#48252=CARTESIAN_POINT ( 'NONE',  ( -11.25000000000000000, 12.50000000000000000, -7.253104124594887736 ) ) ;
#48253=EDGE_CURVE ( 'NONE', #4956, #46788, #98497, .T. ) ;
#48254=ADVANCED_FACE ( 'NONE', ( #21237 ), #50213, .T. ) ;
#48255=DIRECTION ( 'NONE',  ( 0.000000000000000000, 1.000000000000000000, 0.000000000000000000 ) ) ;
#48257=EDGE_CURVE ( 'NONE', #41439, #59702, #12626, .T. ) ;
#48258=CARTESIAN_POINT ( 'NONE',  ( 6.649999999999930189, 2.500000000000000000, 7.088010851410848190 ) ) ;
#48259=AXIS2_PLACEMENT_3D ( 'NONE', #128427, #28923, #19064 ) ;
#48260=VERTEX_POINT ( 'NONE', #89973 ) ;
#48261=AXIS2_PLACEMENT_3D ( 'NONE', #120174, #1669, #41634 ) ;
#48262=EDGE_CURVE ( 'NONE', #55743, #594, #46094, .T. ) ;
#48263=DIRECTION ( 'NONE',  ( -0.000000000000000000, -1.000000000000000000, -0.000000000000000000 ) ) ;
#48264=ORIENTED_EDGE ( 'NONE', *, *, #19506, .T. ) ;
#48265=CARTESIAN_POINT ( 'NONE',  ( -1.450000000000036371, 2.500000000000000000, 2.411473670974873862 ) ) ;
#48266=CARTESIAN_POINT ( 'NONE',  ( 14.93814515115567865, -2.500000000000000444, -6.173787963789434841 ) ) ;
#48267=CARTESIAN_POINT ( 'NONE',  ( 18.20334136264090574, 2.532871263997065636, 4.817802756304448764 ) ) ;
#48268=CARTESIAN_POINT ( 'NONE',  ( -4.600000000000024514, 12.50000000000000000, 3.637306695894644726 ) ) ;
#48269=EDGE_CURVE ( 'NONE', #113705, #77714, #125500, .T. ) ;
#48270=FACE_OUTER_BOUND ( 'NONE', #36132, .T. ) ;
#48271=AXIS2_PLACEMENT_3D ( 'NONE', #46989, #67898, #16832 ) ;
#48272=EDGE_CURVE ( 'NONE', #101260, #91108, #119431, .T. ) ;
#48274=AXIS2_PLACEMENT_3D ( 'NONE', #125782, #96324, #76063 ) ;
#48275=ADVANCED_FACE ( 'NONE', ( #99170 ), #20609, .T. ) ;
#48276=EDGE_CURVE ( 'NONE', #27106, #113976, #69062, .T. ) ;
#48277=VERTEX_POINT ( 'NONE', #120099 ) ;
#48278=ORIENTED_EDGE ( 'NONE', *, *, #6194, .F. ) ;
#48279=ORIENTED_EDGE ( 'NONE', *, *, #34811, .F. ) ;
#48280=ORIENTED_EDGE ( 'NONE', *, *, #41521, .T. ) ;
#48281=FACE_OUTER_BOUND ( 'NONE', #65810, .T. ) ;
#48282=DIRECTION ( 'NONE',  ( -0.000000000000000000, -1.000000000000000000, -0.000000000000000000 ) ) ;
#48283=FACE_OUTER_BOUND ( 'NONE', #53335, .T. ) ;
#48284=FACE_BOUND ( 'NONE', #93639, .T. ) ;
#48285=CARTESIAN_POINT ( 'NONE',  ( -1.450000000000035039, 12.50000000000000000, -2.511473670974877948 ) ) ;
#48286=DIRECTION ( 'NONE',  ( -0.000000000000000000, 1.000000000000000000, -0.000000000000000000 ) ) ;
#48287=EDGE_CURVE ( 'NONE', #83720, #86121, #956, .T. ) ;
#48288=FACE_OUTER_BOUND ( 'NONE', #84963, .T. ) ;
#48289=DIRECTION ( 'NONE',  ( 0.000000000000000000, 0.000000000000000000, 1.000000000000000000 ) ) ;
#48290=AXIS2_PLACEMENT_3D ( 'NONE', #1884, #12347, #53581 ) ;
#48291=AXIS2_PLACEMENT_3D ( 'NONE', #75629, #43631, #46185 ) ;
#48293=DIRECTION ( 'NONE',  ( 0.000000000000000000, 0.000000000000000000, -1.000000000000000000 ) ) ;
#48294=CARTESIAN_POINT ( 'NONE',  ( -1.650000000000034328, 2.500000000000000000, -2.165063509461101710 ) ) ;
#48295=CONICAL_SURFACE ( 'NONE', #121440, 0.09999999999999982514, 0.003490658503988666988 ) ;
#48296=FACE_OUTER_BOUND ( 'NONE', #8206, .T. ) ;
#48298=AXIS2_PLACEMENT_3D ( 'NONE', #123321, #52015, #93862 ) ;
#48299=ORIENTED_EDGE ( 'NONE', *, *, #39706, .T. ) ;
#48300=VERTEX_POINT ( 'NONE', #110899 ) ;
#48301=EDGE_LOOP ( 'NONE', ( #107340, #33396 ) ) ;
#48302=DIRECTION ( 'NONE',  ( 0.000000000000000000, -0.000000000000000000, 1.000000000000000000 ) ) ;
#48303=EDGE_CURVE ( 'NONE', #72180, #4130, #61171, .T. ) ;
#48304=FACE_BOUND ( 'NONE', #33056, .T. ) ;
#48305=CARTESIAN_POINT ( 'NONE',  ( -8.100000000000013856, 12.50000000000000000, -4.741630453620015118 ) ) ;
#48306=ORIENTED_EDGE ( 'NONE', *, *, #7555, .F. ) ;
#48307=FACE_OUTER_BOUND ( 'NONE', #122275, .T. ) ;
#48309=DIRECTION ( 'NONE',  ( -0.000000000000000000, -1.000000000000000000, -0.000000000000000000 ) ) ;
#48310=DIRECTION ( 'NONE',  ( 0.000000000000000000, 0.000000000000000000, 1.000000000000000000 ) ) ;
#48311=EDGE_LOOP ( 'NONE', ( #13031, #60879, #122369, #52991 ) ) ;
#48313=CARTESIAN_POINT ( 'NONE',  ( 17.50000000000000000, 2.500000000000000000, -2.922290670089280340 ) ) ;
#48314=ADVANCED_FACE ( 'NONE', ( #43478 ), #58618, .T. ) ;
#48315=ORIENTED_EDGE ( 'NONE', *, *, #75454, .F. ) ;
#48316=ORIENTED_EDGE ( 'NONE', *, *, #44375, .T. ) ;
#48317=AXIS2_PLACEMENT_3D ( 'NONE', #27592, #76717, #96999 ) ;
#48318=CARTESIAN_POINT ( 'NONE',  ( -7.100000000000017408, 2.500000000000000000, -3.637306695894650055 ) ) ;
#48319=CONICAL_SURFACE ( 'NONE', #81757, 0.09999999999999982514, 0.003490658503988666988 ) ;
#48320=FACE_OUTER_BOUND ( 'NONE', #10064, .T. ) ;
#48321=ORIENTED_EDGE ( 'NONE', *, *, #97288, .F. ) ;
#48322=CARTESIAN_POINT ( 'NONE',  ( 12.89999999999989733, 2.500000000000000000, -2.385244779468109755E-15 ) ) ;
#48323=CIRCLE ( 'NONE', #60848, 0.09999999999999982514 ) ;
#48324=DIRECTION ( 'NONE',  ( 0.000000000000000000, 1.000000000000000000, 0.000000000000000000 ) ) ;
#48325=ORIENTED_EDGE ( 'NONE', *, *, #94169, .T. ) ;
#48326=DIRECTION ( 'NONE',  ( -0.000000000000000000, -1.000000000000000000, -0.000000000000000000 ) ) ;
#48327=ORIENTED_EDGE ( 'NONE', *, *, #111770, .T. ) ;
#48328=CIRCLE ( 'NONE', #91541, 0.1000000000000002554 ) ;
#48329=EDGE_LOOP ( 'NONE', ( #87054, #34190, #125213, #28387 ) ) ;
#48330=EDGE_CURVE ( 'NONE', #14341, #68963, #104316, .T. ) ;
#48331=DIRECTION ( 'NONE',  ( -0.000000000000000000, 1.000000000000000000, -0.000000000000000000 ) ) ;
#48332=ORIENTED_EDGE ( 'NONE', *, *, #56500, .T. ) ;
#48333=CARTESIAN_POINT ( 'NONE',  ( 8.349999999999923261, 2.500000000000000000, 2.065063509461097624 ) ) ;
#48334=FACE_BOUND ( 'NONE', #118812, .T. ) ;
#48335=ORIENTED_EDGE ( 'NONE', *, *, #95642, .T. ) ;
#48337=ORIENTED_EDGE ( 'NONE', *, *, #29650, .T. ) ;
#48338=CARTESIAN_POINT ( 'NONE',  ( -4.600000000000024514, 2.500000000000000000, 5.122947341949749323 ) ) ;
#48339=FACE_OUTER_BOUND ( 'NONE', #102024, .T. ) ;
#48340=FACE_OUTER_BOUND ( 'NONE', #30443, .T. ) ;
#48341=DIRECTION ( 'NONE',  ( 0.000000000000000000, 0.000000000000000000, 1.000000000000000000 ) ) ;
#48343=VERTEX_POINT ( 'NONE', #63098 ) ;
#48344=VERTEX_POINT ( 'NONE', #2230 ) ;
#48345=VERTEX_POINT ( 'NONE', #53929 ) ;
#48346=CARTESIAN_POINT ( 'NONE',  ( 1.249999999999952038, 12.50000000000000000, 5.867463478539781896 ) ) ;
#48347=CARTESIAN_POINT ( 'NONE',  ( -13.54999999999998828, 2.500000000000000000, 1.718653347947325383 ) ) ;
#48349=ORIENTED_EDGE ( 'NONE', *, *, #68001, .T. ) ;
#48350=VERTEX_POINT ( 'NONE', #54552 ) ;
#48351=ORIENTED_EDGE ( 'NONE', *, *, #118536, .T. ) ;
#48352=DIRECTION ( 'NONE',  ( 0.000000000000000000, -0.9999939076577903929, 0.003490651415223739937 ) ) ;
#48353=AXIS2_PLACEMENT_3D ( 'NONE', #24245, #75268, #114541 ) ;
#48354=DIRECTION ( 'NONE',  ( -0.000000000000000000, -1.000000000000000000, -0.000000000000000000 ) ) ;
#48355=AXIS2_PLACEMENT_3D ( 'NONE', #115475, #105690, #66395 ) ;
#48356=ADVANCED_FACE ( 'NONE', ( #12062 ), #62816, .T. ) ;
#48358=DIRECTION ( 'NONE',  ( 0.000000000000000000, 0.000000000000000000, 1.000000000000000000 ) ) ;
#48359=CARTESIAN_POINT ( 'NONE',  ( -14.14999999999998792, 2.500000000000000000, 2.757883832488653209 ) ) ;
#48360=FACE_OUTER_BOUND ( 'NONE', #66691, .T. ) ;
#48361=DIRECTION ( 'NONE',  ( 0.000000000000000000, 0.000000000000000000, 1.000000000000000000 ) ) ;
#48362=CARTESIAN_POINT ( 'NONE',  ( -9.550000000000006040, 2.500000000000000000, 2.265063509461097357 ) ) ;
#48363=DIRECTION ( 'NONE',  ( 0.000000000000000000, 1.000000000000000000, 0.000000000000000000 ) ) ;
#48364=EDGE_CURVE ( 'NONE', #7578, #34866, #77391, .T. ) ;
#48365=ORIENTED_EDGE ( 'NONE', *, *, #51226, .F. ) ;
#48367=EDGE_LOOP ( 'NONE', ( #57164, #59620, #4751, #39184 ) ) ;
#48368=FACE_OUTER_BOUND ( 'NONE', #93569, .T. ) ;
#48369=DIRECTION ( 'NONE',  ( 0.000000000000000000, -0.9999939076577903929, 0.003490651415223739937 ) ) ;
#48370=ADVANCED_FACE ( 'NONE', ( #111555 ), #114138, .T. ) ;
#48371=ORIENTED_EDGE ( 'NONE', *, *, #87512, .T. ) ;
#48373=ORIENTED_EDGE ( 'NONE', *, *, #90892, .T. ) ;
#48374=EDGE_CURVE ( 'NONE', #74697, #111968, #6342, .T. ) ;
#48376=CARTESIAN_POINT ( 'NONE',  ( 13.54999999999989591, 12.50000000000000000, -1.818653347947326138 ) ) ;
#48377=EDGE_CURVE ( 'NONE', #121671, #129577, #37685, .T. ) ;
#48378=CARTESIAN_POINT ( 'NONE',  ( 8.749999999999921840, 2.500000000000000000, 2.957883832488649389 ) ) ;
#48379=CARTESIAN_POINT ( 'NONE',  ( -3.300000000000027800, 12.50000000000000000, -4.330127018922201643 ) ) ;
#48380=AXIS2_PLACEMENT_3D ( 'NONE', #86086, #64533, #4957 ) ;
#48381=CARTESIAN_POINT ( 'NONE',  ( -6.250000000000015987, 2.500000000000000000, 5.902370205355745192 ) ) ;
#48382=LINE ( 'NONE', #107944, #67655 ) ;
#48383=AXIS2_PLACEMENT_3D ( 'NONE', #8948, #69822, #109073 ) ;
#48384=CARTESIAN_POINT ( 'NONE',  ( 6.249999999999967137, 2.500000000000000000, 6.595190528383296780 ) ) ;
#48385=EDGE_CURVE ( 'NONE', #17665, #34432, #110828, .T. ) ;
#48386=AXIS2_PLACEMENT_3D ( 'NONE', #94631, #65159, #86752 ) ;
#48387=CARTESIAN_POINT ( 'NONE',  ( -3.350000000000028955, 12.50000000000000000, 2.165063509461097713 ) ) ;
#48388=EDGE_CURVE ( 'NONE', #113423, #123334, #71121, .T. ) ;
#48389=EDGE_CURVE ( 'NONE', #98382, #51072, #87836, .T. ) ;
#48390=EDGE_LOOP ( 'NONE', ( #115647, #45162 ) ) ;
#48391=AXIS2_PLACEMENT_3D ( 'NONE', #97083, #55860, #26420 ) ;
#48392=AXIS2_PLACEMENT_3D ( 'NONE', #94723, #44998, #102608 ) ;
#48393=VERTEX_POINT ( 'NONE', #64385 ) ;
#48394=EDGE_LOOP ( 'NONE', ( #10076, #19080 ) ) ;
#48396=CARTESIAN_POINT ( 'NONE',  ( 3.749999999999976907, 2.500000000000000000, 2.065063509461097624 ) ) ;
#48397=DIRECTION ( 'NONE',  ( 0.000000000000000000, -0.000000000000000000, 1.000000000000000000 ) ) ;
#48398=ORIENTED_EDGE ( 'NONE', *, *, #112154, .T. ) ;
#48399=DIRECTION ( 'NONE',  ( 0.000000000000000000, -0.9999939076577903929, 0.003490651415223739937 ) ) ;
#48400=CARTESIAN_POINT ( 'NONE',  ( 13.94999999999989271, 2.500000000000000000, -1.718653347947326049 ) ) ;
#48401=DIRECTION ( 'NONE',  ( 0.000000000000000000, 0.000000000000000000, 1.000000000000000000 ) ) ;
#48402=CARTESIAN_POINT ( 'NONE',  ( -12.49999999999995914, 12.50000000000000000, -4.330127018922198978 ) ) ;
#48403=ORIENTED_EDGE ( 'NONE', *, *, #79605, .T. ) ;
#48404=CARTESIAN_POINT ( 'NONE',  ( 12.09999999999990550, 2.500000000000000000, -5.022947341949754119 ) ) ;
#48405=CARTESIAN_POINT ( 'NONE',  ( 2.499999999999981792, 2.500000000000000000, 4.430127018922196847 ) ) ;
#48406=ORIENTED_EDGE ( 'NONE', *, *, #31681, .T. ) ;
#48407=ORIENTED_EDGE ( 'NONE', *, *, #3494, .F. ) ;
#48408=ORIENTED_EDGE ( 'NONE', *, *, #55626, .F. ) ;
#48409=CONICAL_SURFACE ( 'NONE', #21303, 0.09999999999999982514, 0.003490658503988666988 ) ;
#48410=DIRECTION ( 'NONE',  ( 0.000000000000000000, -0.000000000000000000, 1.000000000000000000 ) ) ;
#48411=CIRCLE ( 'NONE', #27552, 0.1000000000000002554 ) ;
#48412=CIRCLE ( 'NONE', #61016, 0.06509327318403743123 ) ;
#48413=CARTESIAN_POINT ( 'NONE',  ( 12.49999999999990408, 2.500000000000000000, -3.637306695894650055 ) ) ;
#48414=CIRCLE ( 'NONE', #23357, 0.06509327318403743123 ) ;
#48415=CIRCLE ( 'NONE', #58795, 0.1000000000000000472 ) ;
#48416=AXIS2_PLACEMENT_3D ( 'NONE', #20654, #100486, #32429 ) ;
#48417=EDGE_LOOP ( 'NONE', ( #120136, #83448 ) ) ;
#48418=DIRECTION ( 'NONE',  ( 0.000000000000000000, 0.000000000000000000, -1.000000000000000000 ) ) ;
#48419=DIRECTION ( 'NONE',  ( 0.000000000000000000, -0.000000000000000000, 1.000000000000000000 ) ) ;
#48420=DIRECTION ( 'NONE',  ( 0.000000000000000000, 0.000000000000000000, 1.000000000000000000 ) ) ;
#48421=DIRECTION ( 'NONE',  ( -0.000000000000000000, -1.000000000000000000, -0.000000000000000000 ) ) ;
#48422=EDGE_CURVE ( 'NONE', #77184, #47267, #104574, .T. ) ;
#48423=CIRCLE ( 'NONE', #123709, 0.06509327318403745899 ) ;
#48425=VERTEX_POINT ( 'NONE', #22554 ) ;
#48426=CARTESIAN_POINT ( 'NONE',  ( 4.399999999999940847, 2.500000000000000000, -3.983716857408426293 ) ) ;
#48427=EDGE_CURVE ( 'NONE', #1725, #114203, #64854, .T. ) ;
#48428=ORIENTED_EDGE ( 'NONE', *, *, #122437, .F. ) ;
#48429=ORIENTED_EDGE ( 'NONE', *, *, #119582, .T. ) ;
#48430=DIRECTION ( 'NONE',  ( 0.000000000000000000, 0.000000000000000000, -1.000000000000000000 ) ) ;
#48431=CARTESIAN_POINT ( 'NONE',  ( -0.8500000000000386136, 12.50000000000000000, 1.407149913249508000 ) ) ;
#48432=FACE_BOUND ( 'NONE', #8100, .T. ) ;
#48433=CARTESIAN_POINT ( 'NONE',  ( 10.64999999999990976, 2.500000000000000000, -6.148780366869526226 ) ) ;
#48434=CARTESIAN_POINT ( 'NONE',  ( 5.849999999999935696, 2.500000000000000000, -7.188010851410854052 ) ) ;
#48435=EDGE_CURVE ( 'NONE', #80189, #11772, #2166, .T. ) ;
#48436=CARTESIAN_POINT ( 'NONE',  ( -1.850000000000033396, 2.500000000000000000, -6.841600689897077814 ) ) ;
#48437=ORIENTED_EDGE ( 'NONE', *, *, #49530, .F. ) ;
#48438=DIRECTION ( 'NONE',  ( 0.000000000000000000, 1.000000000000000000, 0.000000000000000000 ) ) ;
#48439=DIRECTION ( 'NONE',  ( -0.000000000000000000, -1.000000000000000000, -0.000000000000000000 ) ) ;
#48440=LINE ( 'NONE', #49754, #77973 ) ;
#48441=CARTESIAN_POINT ( 'NONE',  ( -3.350000000000031619, 2.500000000000000000, -7.088010851410853519 ) ) ;
#48442=ORIENTED_EDGE ( 'NONE', *, *, #114050, .F. ) ;
#48443=AXIS2_PLACEMENT_3D ( 'NONE', #73832, #74482, #103942 ) ;
#48444=LINE ( 'NONE', #117810, #996 ) ;
#48446=ORIENTED_EDGE ( 'NONE', *, *, #109523, .F. ) ;
#48447=ORIENTED_EDGE ( 'NONE', *, *, #128860, .F. ) ;
#48448=DIRECTION ( 'NONE',  ( 0.000000000000000000, -0.9999939076577903929, 0.003490651415223739937 ) ) ;
#48449=DIRECTION ( 'NONE',  ( 0.000000000000000000, -0.9999939076577903929, 0.003490651415223739937 ) ) ;
#48450=EDGE_CURVE ( 'NONE', #40507, #46262, #108768, .T. ) ;
#48451=FACE_BOUND ( 'NONE', #13044, .T. ) ;
#48452=CIRCLE ( 'NONE', #27498, 0.1000000000000002554 ) ;
#48453=DIRECTION ( 'NONE',  ( -4.274815082592931898E-19, -0.9999939076577903929, -0.003490651415223739937 ) ) ;
#48454=CIRCLE ( 'NONE', #407, 0.06509327318403745899 ) ;
#48455=AXIS2_PLACEMENT_3D ( 'NONE', #14918, #96092, #84978 ) ;
#48456=ORIENTED_EDGE ( 'NONE', *, *, #78405, .F. ) ;
#48457=CONICAL_SURFACE ( 'NONE', #67497, 0.1000000000000002554, 0.003490658503988666988 ) ;
#48458=CARTESIAN_POINT ( 'NONE',  ( 1.899999999999951283, 12.50000000000000000, -3.983716857408426293 ) ) ;
#48459=VECTOR ( 'NONE', #84553, 1000.000000000000000 ) ;
#48460=ORIENTED_EDGE ( 'NONE', *, *, #88580, .T. ) ;
#48461=ORIENTED_EDGE ( 'NONE', *, *, #25363, .T. ) ;
#48462=CARTESIAN_POINT ( 'NONE',  ( 3.949999999999939782, 2.500000000000000000, 2.511473670974873507 ) ) ;
#48464=ORIENTED_EDGE ( 'NONE', *, *, #104111, .T. ) ;
#48465=CIRCLE ( 'NONE', #90214, 0.1000000000000002554 ) ;
#48466=CARTESIAN_POINT ( 'NONE',  ( -9.150000000000009237, 2.500000000000000000, -6.595190528383296780 ) ) ;
#48468=CIRCLE ( 'NONE', #115340, 0.06509327318403745899 ) ;
#48469=EDGE_CURVE ( 'NONE', #23517, #15869, #67306, .T. ) ;
#48470=CONICAL_SURFACE ( 'NONE', #65168, 0.1000000000000000472, 0.003490658503988666988 ) ;
#48471=AXIS2_PLACEMENT_3D ( 'NONE', #104852, #15170, #123230 ) ;
#48472=AXIS2_PLACEMENT_3D ( 'NONE', #46227, #107068, #116250 ) ;
#48473=DIRECTION ( 'NONE',  ( 0.000000000000000000, 0.000000000000000000, 1.000000000000000000 ) ) ;
#48474=DIRECTION ( 'NONE',  ( 0.000000000000000000, 0.000000000000000000, 1.000000000000000000 ) ) ;
#48475=ORIENTED_EDGE ( 'NONE', *, *, #62702, .T. ) ;
#48476=CARTESIAN_POINT ( 'NONE',  ( -10.85000000000000142, 2.500000000000000000, 2.165063509461097713 ) ) ;
#48477=CIRCLE ( 'NONE', #19219, 0.1000000000000002554 ) ;
#48478=FACE_OUTER_BOUND ( 'NONE', #73482, .T. ) ;
#48479=CARTESIAN_POINT ( 'NONE',  ( -9.400000000000009237, 12.50000000000000000, -3.983716857408421852 ) ) ;
#48481=ORIENTED_EDGE ( 'NONE', *, *, #26374, .F. ) ;
#48482=CARTESIAN_POINT ( 'NONE',  ( 6.249999999999930722, 12.50000000000000000, 1.472243186433545459 ) ) ;
#48483=ORIENTED_EDGE ( 'NONE', *, *, #81076, .T. ) ;
#48484=EDGE_CURVE ( 'NONE', #1730, #50100, #125872, .T. ) ;
#48485=CARTESIAN_POINT ( 'NONE',  ( 7.499999999999925393, 2.500000000000000000, 5.022947341949748790 ) ) ;
#48486=VERTEX_POINT ( 'NONE', #17858 ) ;
#48487=DIRECTION ( 'NONE',  ( 0.000000000000000000, 0.000000000000000000, -1.000000000000000000 ) ) ;
#48488=PLANE ( 'NONE',  #24348 ) ;
#48489=DIRECTION ( 'NONE',  ( -4.274815082592931898E-19, -0.9999939076577903929, -0.003490651415223739937 ) ) ;
#48490=DIRECTION ( 'NONE',  ( 0.000000000000000000, 0.000000000000000000, 1.000000000000000000 ) ) ;
#48491=ORIENTED_EDGE ( 'NONE', *, *, #128451, .T. ) ;
#48492=DIRECTION ( 'NONE',  ( -0.000000000000000000, -1.000000000000000000, -0.000000000000000000 ) ) ;
#48493=FACE_OUTER_BOUND ( 'NONE', #26278, .T. ) ;
#48494=LINE ( 'NONE', #38705, #21397 ) ;
#48495=EDGE_CURVE ( 'NONE', #92739, #123569, #121621, .T. ) ;
#48496=PLANE ( 'NONE',  #26562 ) ;
#48497=DIRECTION ( 'NONE',  ( -0.000000000000000000, 1.000000000000000000, -0.000000000000000000 ) ) ;
#48498=CARTESIAN_POINT ( 'NONE',  ( -5.850000000000018296, 2.500000000000000000, 7.288010851410849256 ) ) ;
#48499=ORIENTED_EDGE ( 'NONE', *, *, #67430, .T. ) ;
#48500=ORIENTED_EDGE ( 'NONE', *, *, #83457, .F. ) ;
#48501=LINE ( 'NONE', #47872, #63817 ) ;
#48502=ORIENTED_EDGE ( 'NONE', *, *, #86480, .F. ) ;
#48503=AXIS2_PLACEMENT_3D ( 'NONE', #10906, #61985, #29303 ) ;
#48504=DIRECTION ( 'NONE',  ( -0.000000000000000000, -1.000000000000000000, -0.000000000000000000 ) ) ;
#48505=AXIS2_PLACEMENT_3D ( 'NONE', #6688, #47304, #77404 ) ;
#48506=AXIS2_PLACEMENT_3D ( 'NONE', #80581, #59673, #11173 ) ;
#48507=ORIENTED_EDGE ( 'NONE', *, *, #111458, .T. ) ;
#48508=EDGE_LOOP ( 'NONE', ( #39130, #78786, #108101, #33432 ) ) ;
#48509=VERTEX_POINT ( 'NONE', #34951 ) ;
#48510=CARTESIAN_POINT ( 'NONE',  ( 1.049999999999953637, 2.500000000000000000, -1.918653347947326004 ) ) ;
#48511=DIRECTION ( 'NONE',  ( -0.000000000000000000, -1.000000000000000000, -0.000000000000000000 ) ) ;
#48512=CONICAL_SURFACE ( 'NONE', #23463, 0.09999999999999982514, 0.003490658503988666988 ) ;
#48513=AXIS2_PLACEMENT_3D ( 'NONE', #86380, #15035, #56276 ) ;
#48515=CIRCLE ( 'NONE', #50550, 0.09999999999999999167 ) ;
#48516=EDGE_CURVE ( 'NONE', #97511, #36170, #116701, .T. ) ;
#48517=DIRECTION ( 'NONE',  ( 0.000000000000000000, -0.000000000000000000, 1.000000000000000000 ) ) ;
#48518=DIRECTION ( 'NONE',  ( -0.000000000000000000, -1.000000000000000000, -0.000000000000000000 ) ) ;
#48519=AXIS2_PLACEMENT_3D ( 'NONE', #65055, #103065, #13390 ) ;
#48521=CARTESIAN_POINT ( 'NONE',  ( -9.150000000000005684, 2.500000000000000000, 7.188010851410848723 ) ) ;
#48522=VECTOR ( 'NONE', #87206, 1000.000000000000000 ) ;
#48523=LINE ( 'NONE', #88431, #110507 ) ;
#48524=EDGE_LOOP ( 'NONE', ( #22325, #128470 ) ) ;
#48525=EDGE_CURVE ( 'NONE', #69489, #126455, #65008, .T. ) ;
#48526=ORIENTED_EDGE ( 'NONE', *, *, #67223, .F. ) ;
#48527=VERTEX_POINT ( 'NONE', #25750 ) ;
#48528=DIRECTION ( 'NONE',  ( 0.000000000000000000, 1.000000000000000000, 0.000000000000000000 ) ) ;
#48529=EDGE_CURVE ( 'NONE', #12380, #78590, #88149, .T. ) ;
#48530=EDGE_LOOP ( 'NONE', ( #105757, #67798 ) ) ;
#48531=EDGE_CURVE ( 'NONE', #1733, #91438, #50614, .T. ) ;
#48532=VERTEX_POINT ( 'NONE', #7386 ) ;
#48533=ADVANCED_FACE ( 'NONE', ( #116061 ), #48470, .T. ) ;
#48534=CARTESIAN_POINT ( 'NONE',  ( 13.34999999999990017, 2.500000000000000000, 1.572243186433545548 ) ) ;
#48535=EDGE_CURVE ( 'NONE', #384, #91010, #113305, .T. ) ;
#48536=DIRECTION ( 'NONE',  ( 0.000000000000000000, 0.000000000000000000, 1.000000000000000000 ) ) ;
#48537=DIRECTION ( 'NONE',  ( 0.000000000000000000, 1.000000000000000000, 0.000000000000000000 ) ) ;
#48539=DIRECTION ( 'NONE',  ( 0.000000000000000000, 0.000000000000000000, 1.000000000000000000 ) ) ;
#48540=ADVANCED_FACE ( 'NONE', ( #46686 ), #45407, .T. ) ;
#48541=DIRECTION ( 'NONE',  ( 0.000000000000000000, 0.000000000000000000, 1.000000000000000000 ) ) ;
#48542=ORIENTED_EDGE ( 'NONE', *, *, #59637, .T. ) ;
#48543=EDGE_CURVE ( 'NONE', #16181, #120910, #95144, .T. ) ;
#48544=ADVANCED_FACE ( 'NONE', ( #96409 ), #105613, .T. ) ;
#48545=PLANE ( 'NONE',  #122408 ) ;
#48546=EDGE_CURVE ( 'NONE', #38970, #82397, #67597, .T. ) ;
#48547=VERTEX_POINT ( 'NONE', #27048 ) ;
#48548=CARTESIAN_POINT ( 'NONE',  ( 15.19999999999989271, 2.500000000000000000, -0.3464101615137783474 ) ) ;
#48549=EDGE_CURVE ( 'NONE', #19084, #53181, #96566, .T. ) ;
#48550=EDGE_LOOP ( 'NONE', ( #54235, #98065 ) ) ;
#48551=CARTESIAN_POINT ( 'NONE',  ( 3.749999999999944045, 2.500000000000000000, -7.088010851410853519 ) ) ;
#48552=EDGE_LOOP ( 'NONE', ( #85717, #128853 ) ) ;
#48554=EDGE_CURVE ( 'NONE', #37632, #103010, #117480, .T. ) ;
#48555=CARTESIAN_POINT ( 'NONE',  ( -7.900000000000011013, 12.50000000000000000, 4.957854068765711553 ) ) ;
#48556=DIRECTION ( 'NONE',  ( 0.000000000000000000, 1.000000000000000000, 0.000000000000000000 ) ) ;
#48557=AXIS2_PLACEMENT_3D ( 'NONE', #112126, #70264, #59829 ) ;
#48558=VECTOR ( 'NONE', #40029, 1000.000000000000000 ) ;
#48559=CARTESIAN_POINT ( 'NONE',  ( 11.04999999999990656, 2.500000000000000000, -6.248780366869526759 ) ) ;
#48560=AXIS2_PLACEMENT_3D ( 'NONE', #110373, #60651, #112318 ) ;
#48561=FACE_OUTER_BOUND ( 'NONE', #59751, .T. ) ;
#48563=ORIENTED_EDGE ( 'NONE', *, *, #60748, .T. ) ;
#48564=CARTESIAN_POINT ( 'NONE',  ( -4.600000000000024514, 2.500000000000000000, -0.7928203230275543412 ) ) ;
#48565=CARTESIAN_POINT ( 'NONE',  ( 13.09999999999990195, 12.50000000000000000, 4.676537180435972552 ) ) ;
#48566=FACE_OUTER_BOUND ( 'NONE', #71760, .T. ) ;
#48567=DIRECTION ( 'NONE',  ( -0.000000000000000000, 1.000000000000000000, -0.000000000000000000 ) ) ;
#48568=CONICAL_SURFACE ( 'NONE', #123750, 0.1000000000000002554, 0.003490658503988666988 ) ;
#48570=CARTESIAN_POINT ( 'NONE',  ( 1.649999999999950617, 2.500000000000000000, -2.065063509461102065 ) ) ;
#48571=ORIENTED_EDGE ( 'NONE', *, *, #52107, .T. ) ;
#48572=CONICAL_SURFACE ( 'NONE', #102938, 0.1000000000000002554, 0.003490658503988666988 ) ;
#48573=VECTOR ( 'NONE', #104695, 1000.000000000000000 ) ;
#48574=CONICAL_SURFACE ( 'NONE', #2566, 0.09999999999999982514, 0.003490658503988666988 ) ;
#48575=VERTEX_POINT ( 'NONE', #66946 ) ;
#48576=DIRECTION ( 'NONE',  ( 0.000000000000000000, 1.000000000000000000, 0.000000000000000000 ) ) ;
#48577=CIRCLE ( 'NONE', #6674, 0.06509327318403745899 ) ;
#48578=ORIENTED_EDGE ( 'NONE', *, *, #97204, .T. ) ;
#48579=FACE_OUTER_BOUND ( 'NONE', #38579, .T. ) ;
#48580=DIRECTION ( 'NONE',  ( -0.000000000000000000, 1.000000000000000000, -0.000000000000000000 ) ) ;
#48581=CONICAL_SURFACE ( 'NONE', #92484, 0.1000000000000002554, 0.003490658503988666988 ) ;
#48582=ORIENTED_EDGE ( 'NONE', *, *, #35980, .F. ) ;
#48584=DIRECTION ( 'NONE',  ( 0.000000000000000000, 0.000000000000000000, -1.000000000000000000 ) ) ;
#48585=LINE ( 'NONE', #16518, #77477 ) ;
#48586=CARTESIAN_POINT ( 'NONE',  ( -1.450000000000035039, 2.500000000000000000, -6.841600689897077814 ) ) ;
#48587=EDGE_LOOP ( 'NONE', ( #92582, #20587, #58909, #124379 ) ) ;
#48588=EDGE_CURVE ( 'NONE', #10139, #41152, #35952, .T. ) ;
#48589=DIRECTION ( 'NONE',  ( 0.000000000000000000, 1.000000000000000000, 0.000000000000000000 ) ) ;
#48590=EDGE_CURVE ( 'NONE', #105322, #119917, #117317, .T. ) ;
#48591=VERTEX_POINT ( 'NONE', #107540 ) ;
#48592=CARTESIAN_POINT ( 'NONE',  ( 10.19999999999991047, 12.50000000000000000, 4.676537180435972552 ) ) ;
#48593=CARTESIAN_POINT ( 'NONE',  ( 5.399999999999936406, 2.500000000000000000, -5.122947341949753763 ) ) ;
#48594=CARTESIAN_POINT ( 'NONE',  ( 11.24999999999990763, 2.500000000000000000, -7.288010851410854585 ) ) ;
#48595=EDGE_CURVE ( 'NONE', #22696, #98598, #57802, .T. ) ;
#48596=ORIENTED_EDGE ( 'NONE', *, *, #45504, .F. ) ;
#48597=CARTESIAN_POINT ( 'NONE',  ( -13.74999999999998757, 2.500000000000000000, 1.472243186433549456 ) ) ;
#48598=AXIS2_PLACEMENT_3D ( 'NONE', #13050, #32095, #23533 ) ;
#48599=VECTOR ( 'NONE', #77826, 1000.000000000000000 ) ;
#48600=VERTEX_POINT ( 'NONE', #124607 ) ;
#48601=CARTESIAN_POINT ( 'NONE',  ( 5.649999999999932854, 12.50000000000000000, 1.818653347947321475 ) ) ;
#48603=DIRECTION ( 'NONE',  ( 0.000000000000000000, 0.000000000000000000, 1.000000000000000000 ) ) ;
#48604=VERTEX_POINT ( 'NONE', #50536 ) ;
#48605=CIRCLE ( 'NONE', #15114, 0.09999999999999982514 ) ;
#48606=CARTESIAN_POINT ( 'NONE',  ( -9.800000000000006040, 2.500000000000000000, 4.776537180435972196 ) ) ;
#48607=AXIS2_PLACEMENT_3D ( 'NONE', #60799, #109237, #129570 ) ;
#48608=LINE ( 'NONE', #9318, #32837 ) ;
#48609=CIRCLE ( 'NONE', #104924, 0.1000000000000002554 ) ;
#48610=VERTEX_POINT ( 'NONE', #109472 ) ;
#48611=AXIS2_PLACEMENT_3D ( 'NONE', #66696, #94878, #5191 ) ;
#48612=DIRECTION ( 'NONE',  ( 0.000000000000000000, 1.000000000000000000, 0.000000000000000000 ) ) ;
#48613=ORIENTED_EDGE ( 'NONE', *, *, #20634, .F. ) ;
#48614=CARTESIAN_POINT ( 'NONE',  ( -4.150000000000025224, 2.500000000000000000, 2.857883832488649301 ) ) ;
#48615=EDGE_LOOP ( 'NONE', ( #83986, #11850, #77320, #9773 ) ) ;
#48617=CARTESIAN_POINT ( 'NONE',  ( -6.249999999999984901, 12.50000000000000000, -6.560283801567339701 ) ) ;
#48618=VERTEX_POINT ( 'NONE', #70832 ) ;
#48619=ORIENTED_EDGE ( 'NONE', *, *, #55037, .T. ) ;
#48620=DIRECTION ( 'NONE',  ( 0.000000000000000000, 0.000000000000000000, 1.000000000000000000 ) ) ;
#48621=CARTESIAN_POINT ( 'NONE',  ( 11.24999999999990941, 12.50000000000000000, -1.537336459617587581 ) ) ;
#48622=ORIENTED_EDGE ( 'NONE', *, *, #60248, .F. ) ;
#48623=CIRCLE ( 'NONE', #44505, 0.1000000000000002554 ) ;
#48624=CARTESIAN_POINT ( 'NONE',  ( 10.64999999999991331, 2.500000000000000000, -2.611473670974877592 ) ) ;
#48625=EDGE_CURVE ( 'NONE', #52844, #54614, #100770, .T. ) ;
#48626=CARTESIAN_POINT ( 'NONE',  ( -13.94999999999998685, 2.500000000000000000, -2.511473670974875727 ) ) ;
#48627=FACE_OUTER_BOUND ( 'NONE', #94046, .T. ) ;
#48629=DIRECTION ( 'NONE',  ( 0.000000000000000000, 0.000000000000000000, 1.000000000000000000 ) ) ;
#48630=DIRECTION ( 'NONE',  ( 0.000000000000000000, 1.000000000000000000, 0.000000000000000000 ) ) ;
#48631=CARTESIAN_POINT ( 'NONE',  ( -10.80000000000000071, 12.50000000000000000, 4.395220292106234439 ) ) ;
#48632=EDGE_LOOP ( 'NONE', ( #20610, #19168, #85086, #94173 ) ) ;
#48633=VERTEX_POINT ( 'NONE', #38831 ) ;
#48634=EDGE_LOOP ( 'NONE', ( #59900, #106493 ) ) ;
#48635=ORIENTED_EDGE ( 'NONE', *, *, #126225, .F. ) ;
#48636=CARTESIAN_POINT ( 'NONE',  ( -3.350000000000029399, 12.50000000000000000, 6.560283801567334372 ) ) ;
#48637=DIRECTION ( 'NONE',  ( 0.000000000000000000, 0.000000000000000000, 1.000000000000000000 ) ) ;
#48638=EDGE_CURVE ( 'NONE', #102323, #127947, #44353, .T. ) ;
#48639=CARTESIAN_POINT ( 'NONE',  ( -0.8500000000000395017, 2.500000000000000000, 6.395190528383296602 ) ) ;
#48640=EDGE_LOOP ( 'NONE', ( #90133, #47713, #67779, #37295 ) ) ;
#48641=FACE_BOUND ( 'NONE', #126463, .T. ) ;
#48642=ORIENTED_EDGE ( 'NONE', *, *, #52372, .F. ) ;
#48643=EDGE_CURVE ( 'NONE', #53612, #17715, #73592, .T. ) ;
#48644=CIRCLE ( 'NONE', #75725, 0.09999999999999982514 ) ;
#48645=LINE ( 'NONE', #19154, #50063 ) ;
#48648=AXIS2_PLACEMENT_3D ( 'NONE', #99037, #61039, #68924 ) ;
#48649=LINE ( 'NONE', #18533, #105687 ) ;
#48650=AXIS2_PLACEMENT_3D ( 'NONE', #909, #128605, #29724 ) ;
#48651=DIRECTION ( 'NONE',  ( 0.000000000000000000, 0.000000000000000000, -1.000000000000000000 ) ) ;
#48652=DIRECTION ( 'NONE',  ( 0.000000000000000000, 0.000000000000000000, 1.000000000000000000 ) ) ;
#48653=CARTESIAN_POINT ( 'NONE',  ( -5.450000000000023270, 12.50000000000000000, -6.495190528383302464 ) ) ;
#48654=DIRECTION ( 'NONE',  ( 0.000000000000000000, 1.000000000000000000, 0.000000000000000000 ) ) ;
#48655=DIRECTION ( 'NONE',  ( 0.000000000000000000, 0.000000000000000000, 1.000000000000000000 ) ) ;
#48656=EDGE_CURVE ( 'NONE', #15598, #80232, #71544, .T. ) ;
#48657=CARTESIAN_POINT ( 'NONE',  ( 2.049999999999950084, 2.500000000000000000, -6.595190528383302109 ) ) ;
#48658=CIRCLE ( 'NONE', #121801, 0.06509327318403745899 ) ;
#48659=DIRECTION ( 'NONE',  ( 0.000000000000000000, 0.000000000000000000, 1.000000000000000000 ) ) ;
#48660=VERTEX_POINT ( 'NONE', #11260 ) ;
#48661=EDGE_LOOP ( 'NONE', ( #97904, #33186 ) ) ;
#48662=ORIENTED_EDGE ( 'NONE', *, *, #124499, .F. ) ;
#48663=AXIS2_PLACEMENT_3D ( 'NONE', #79534, #20615, #49445 ) ;
#48664=ORIENTED_EDGE ( 'NONE', *, *, #126116, .T. ) ;
#48665=AXIS2_PLACEMENT_3D ( 'NONE', #37276, #47097, #117731 ) ;
#48666=AXIS2_PLACEMENT_3D ( 'NONE', #55585, #44469, #45130 ) ;
#48667=CARTESIAN_POINT ( 'NONE',  ( -12.89999999999999325, 2.500000000000000000, 0.6928203230275535862 ) ) ;
#48668=DIRECTION ( 'NONE',  ( 0.000000000000000000, 0.000000000000000000, -1.000000000000000000 ) ) ;
#48669=EDGE_LOOP ( 'NONE', ( #105830, #116758, #95158, #77483 ) ) ;
#48670=EDGE_LOOP ( 'NONE', ( #103540, #58676, #44907, #24934 ) ) ;
#48671=VERTEX_POINT ( 'NONE', #18508 ) ;
#48672=AXIS2_PLACEMENT_3D ( 'NONE', #58133, #38505, #99346 ) ;
#48673=DIRECTION ( 'NONE',  ( 0.000000000000000000, 1.000000000000000000, 0.000000000000000000 ) ) ;
#48674=CARTESIAN_POINT ( 'NONE',  ( -8.749999999999971578, 2.500000000000000000, 6.495190528383297135 ) ) ;
#48675=CARTESIAN_POINT ( 'NONE',  ( -9.150000000000009237, 2.500000000000000000, 2.065063509461097624 ) ) ;
#48676=DIRECTION ( 'NONE',  ( 0.000000000000000000, 0.000000000000000000, 1.000000000000000000 ) ) ;
#48677=DIRECTION ( 'NONE',  ( 0.000000000000000000, 0.000000000000000000, -1.000000000000000000 ) ) ;
#48679=CARTESIAN_POINT ( 'NONE',  ( 7.699999999999925571, 2.500000000000000000, 3.883716857408420431 ) ) ;
#48680=ORIENTED_EDGE ( 'NONE', *, *, #85936, .F. ) ;
#48681=CARTESIAN_POINT ( 'NONE',  ( 1.649999999999950617, 2.500000000000000000, 2.165063509461097713 ) ) ;
#48682=EDGE_LOOP ( 'NONE', ( #73029, #57849 ) ) ;
#48683=ADVANCED_FACE ( 'NONE', ( #58453 ), #15074, .T. ) ;
#48684=ORIENTED_EDGE ( 'NONE', *, *, #118875, .T. ) ;
#48685=EDGE_LOOP ( 'NONE', ( #20593, #36652 ) ) ;
#48686=DIRECTION ( 'NONE',  ( 0.000000000000000000, 0.000000000000000000, 1.000000000000000000 ) ) ;
#48687=AXIS2_PLACEMENT_3D ( 'NONE', #68801, #697, #69436 ) ;
#48688=CONICAL_SURFACE ( 'NONE', #19415, 0.1000000000000000472, 0.003490658503988666988 ) ;
#48689=EDGE_LOOP ( 'NONE', ( #81262, #98408 ) ) ;
#48690=EDGE_CURVE ( 'NONE', #119719, #21947, #61089, .T. ) ;
#48691=ORIENTED_EDGE ( 'NONE', *, *, #14090, .F. ) ;
#48692=EDGE_CURVE ( 'NONE', #19521, #104314, #84060, .T. ) ;
#48693=DIRECTION ( 'NONE',  ( -0.000000000000000000, -1.000000000000000000, -0.000000000000000000 ) ) ;
#48694=CARTESIAN_POINT ( 'NONE',  ( 2.099999999999950351, 12.50000000000000000, -0.06509327318403970719 ) ) ;
#48695=DIRECTION ( 'NONE',  ( -0.000000000000000000, 1.000000000000000000, -0.000000000000000000 ) ) ;
#48696=CONICAL_SURFACE ( 'NONE', #75862, 0.1000000000000000056, 0.003490658503988666988 ) ;
#48697=CARTESIAN_POINT ( 'NONE',  ( 14.79999999999989235, 12.50000000000000000, 0.2813168883297361700 ) ) ;
#48699=AXIS2_PLACEMENT_3D ( 'NONE', #103115, #13432, #53382 ) ;
#48700=ADVANCED_FACE ( 'NONE', ( #98345 ), #46402, .T. ) ;
#48701=CARTESIAN_POINT ( 'NONE',  ( -7.500000000000013323, 12.50000000000000000, 4.957854068765711553 ) ) ;
#48702=ADVANCED_FACE ( 'NONE', ( #89187 ), #14988, .T. ) ;
#48703=ORIENTED_EDGE ( 'NONE', *, *, #117512, .T. ) ;
#48704=DIRECTION ( 'NONE',  ( -0.000000000000000000, -1.000000000000000000, -0.000000000000000000 ) ) ;
#48705=AXIS2_PLACEMENT_3D ( 'NONE', #117272, #77385, #99611 ) ;
#48706=AXIS2_PLACEMENT_3D ( 'NONE', #29894, #118264, #30561 ) ;
#48707=EDGE_LOOP ( 'NONE', ( #90925, #71052, #3369, #45090 ) ) ;
#48708=CARTESIAN_POINT ( 'NONE',  ( 5.399999999999931966, 2.500000000000000000, 4.430127018922196847 ) ) ;
#48709=CIRCLE ( 'NONE', #11023, 0.09999999999999982514 ) ;
#48710=EDGE_CURVE ( 'NONE', #18522, #75910, #86098, .T. ) ;
#48711=VERTEX_POINT ( 'NONE', #40092 ) ;
#48712=LINE ( 'NONE', #129223, #66365 ) ;
#48713=DIRECTION ( 'NONE',  ( 0.000000000000000000, 1.000000000000000000, 0.000000000000000000 ) ) ;
#48714=AXIS2_PLACEMENT_3D ( 'NONE', #21125, #21795, #72182 ) ;
#48715=ORIENTED_EDGE ( 'NONE', *, *, #13664, .T. ) ;
#48716=CIRCLE ( 'NONE', #34036, 0.09999999999999982514 ) ;
#48717=DIRECTION ( 'NONE',  ( 0.000000000000000000, -0.9999939076577903929, 0.003490651415223739937 ) ) ;
#48718=CARTESIAN_POINT ( 'NONE',  ( -11.84999999999999787, 12.50000000000000000, -6.776507416713037024 ) ) ;
#48719=ORIENTED_EDGE ( 'NONE', *, *, #98313, .F. ) ;
#48720=EDGE_CURVE ( 'NONE', #82761, #69440, #29615, .T. ) ;
#48721=CIRCLE ( 'NONE', #82052, 0.09999999999999982514 ) ;
#48722=DIRECTION ( 'NONE',  ( -0.000000000000000000, 1.000000000000000000, -0.000000000000000000 ) ) ;
#48723=ORIENTED_EDGE ( 'NONE', *, *, #82875, .T. ) ;
#48724=VERTEX_POINT ( 'NONE', #128492 ) ;
#48725=FACE_OUTER_BOUND ( 'NONE', #50986, .T. ) ;
#48726=DIRECTION ( 'NONE',  ( 0.000000000000000000, 1.000000000000000000, 0.000000000000000000 ) ) ;
#48728=CARTESIAN_POINT ( 'NONE',  ( -4.150000000000025224, 2.500000000000000000, 5.702370205355745014 ) ) ;
#48729=CIRCLE ( 'NONE', #121866, 0.06509327318403741736 ) ;
#48730=DIRECTION ( 'NONE',  ( 0.000000000000000000, 0.000000000000000000, 1.000000000000000000 ) ) ;
#48731=ORIENTED_EDGE ( 'NONE', *, *, #6056, .F. ) ;
#48732=CARTESIAN_POINT ( 'NONE',  ( 9.149999999999918643, 12.50000000000000000, -6.495190528383302464 ) ) ;
#48734=ORIENTED_EDGE ( 'NONE', *, *, #94708, .T. ) ;
#48736=DIRECTION ( 'NONE',  ( 0.000000000000000000, 0.000000000000000000, -1.000000000000000000 ) ) ;
#48737=DIRECTION ( 'NONE',  ( 0.000000000000000000, 0.000000000000000000, 1.000000000000000000 ) ) ;
#48738=AXIS2_PLACEMENT_3D ( 'NONE', #64878, #4652, #43978 ) ;
#48739=ORIENTED_EDGE ( 'NONE', *, *, #89273, .F. ) ;
#48740=DIRECTION ( 'NONE',  ( 0.000000000000000000, 1.000000000000000000, 0.000000000000000000 ) ) ;
#48741=DIRECTION ( 'NONE',  ( 0.000000000000000000, 0.000000000000000000, 1.000000000000000000 ) ) ;
#48742=DIRECTION ( 'NONE',  ( 0.000000000000000000, 1.000000000000000000, 0.000000000000000000 ) ) ;
#48743=CARTESIAN_POINT ( 'NONE',  ( -11.84999999999999609, 2.500000000000000000, 6.248780366869521430 ) ) ;
#48744=CIRCLE ( 'NONE', #54983, 0.1000000000000002554 ) ;
#48745=CARTESIAN_POINT ( 'NONE',  ( -0.6500000000000403233, 2.500000000000000000, 6.048780366869520364 ) ) ;
#48746=CIRCLE ( 'NONE', #113581, 0.1000000000000000472 ) ;
#48747=ORIENTED_EDGE ( 'NONE', *, *, #93619, .F. ) ;
#48748=CIRCLE ( 'NONE', #44525, 0.06509327318403745899 ) ;
#48749=VECTOR ( 'NONE', #40709, 1000.000000000000000 ) ;
#48750=EDGE_CURVE ( 'NONE', #65189, #74144, #79858, .T. ) ;
#48751=CARTESIAN_POINT ( 'NONE',  ( -10.40000000000000213, 2.500000000000000000, -5.022947341949749678 ) ) ;
#48752=CARTESIAN_POINT ( 'NONE',  ( 5.649999999999932854, 12.50000000000000000, 2.511473670974873507 ) ) ;
#48753=AXIS2_PLACEMENT_3D ( 'NONE', #108484, #128807, #8988 ) ;
#48754=VERTEX_POINT ( 'NONE', #110117 ) ;
#48755=DIRECTION ( 'NONE',  ( -0.000000000000000000, -1.000000000000000000, -0.000000000000000000 ) ) ;
#48756=EDGE_CURVE ( 'NONE', #29100, #18148, #4611, .T. ) ;
#48757=VERTEX_POINT ( 'NONE', #40757 ) ;
#48758=CONICAL_SURFACE ( 'NONE', #90499, 0.1000000000000002554, 0.003490658503988666988 ) ;
#48759=CIRCLE ( 'NONE', #44643, 0.06509327318403745899 ) ;
#48760=ORIENTED_EDGE ( 'NONE', *, *, #29847, .T. ) ;
#48762=CIRCLE ( 'NONE', #15273, 0.1000000000000002554 ) ;
#48763=ORIENTED_EDGE ( 'NONE', *, *, #84758, .F. ) ;
#48764=CARTESIAN_POINT ( 'NONE',  ( 9.599999999999914380, 12.50000000000000000, -3.637306695894650055 ) ) ;
#48765=DIRECTION ( 'NONE',  ( -4.274815082592931898E-19, -0.9999939076577903929, -0.003490651415223739937 ) ) ;
#48766=ORIENTED_EDGE ( 'NONE', *, *, #14820, .T. ) ;
#48767=CARTESIAN_POINT ( 'NONE',  ( 12.29999999999990123, 2.500000000000000000, 0.2464101615137735679 ) ) ;
#48768=AXIS2_PLACEMENT_3D ( 'NONE', #27879, #26596, #37706 ) ;
#48769=DIRECTION ( 'NONE',  ( 0.000000000000000000, -0.9999939076577903929, 0.003490651415223739937 ) ) ;
#48770=VERTEX_POINT ( 'NONE', #48621 ) ;
#48771=PLANE ( 'NONE',  #31920 ) ;
#48773=ORIENTED_EDGE ( 'NONE', *, *, #108514, .T. ) ;
#48774=VERTEX_POINT ( 'NONE', #28990 ) ;
#48775=EDGE_LOOP ( 'NONE', ( #109067, #78494, #45399, #32347 ) ) ;
#48776=CARTESIAN_POINT ( 'NONE',  ( -14.14999999999998792, 12.50000000000000000, -1.537336459617585360 ) ) ;
#48777=DIRECTION ( 'NONE',  ( -4.274815082592931898E-19, -0.9999939076577903929, -0.003490651415223739937 ) ) ;
#48778=CIRCLE ( 'NONE', #30001, 0.06509327318403745899 ) ;
#48779=FACE_OUTER_BOUND ( 'NONE', #34296, .T. ) ;
#48780=FACE_BOUND ( 'NONE', #12783, .T. ) ;
#48781=ORIENTED_EDGE ( 'NONE', *, *, #68361, .F. ) ;
#48782=LINE ( 'NONE', #67087, #82496 ) ;
#48783=DIRECTION ( 'NONE',  ( -0.000000000000000000, -1.000000000000000000, -0.000000000000000000 ) ) ;
#48784=VERTEX_POINT ( 'NONE', #80666 ) ;
#48785=CARTESIAN_POINT ( 'NONE',  ( -3.350000000000029399, 2.500000000000000000, 6.595190528383296780 ) ) ;
#48786=ADVANCED_FACE ( 'NONE', ( #68895 ), #33897, .T. ) ;
#48787=CIRCLE ( 'NONE', #121940, 2.000000000000000000 ) ;
#48789=CONICAL_SURFACE ( 'NONE', #44575, 0.09999999999999982514, 0.003490658503988666988 ) ;
#48790=DIRECTION ( 'NONE',  ( 0.000000000000000000, 0.000000000000000000, 1.000000000000000000 ) ) ;
#48791=CIRCLE ( 'NONE', #119884, 0.1000000000000002554 ) ;
#48792=FACE_OUTER_BOUND ( 'NONE', #39761, .T. ) ;
#48793=DIRECTION ( 'NONE',  ( 0.000000000000000000, 0.000000000000000000, 1.000000000000000000 ) ) ;
#48794=DIRECTION ( 'NONE',  ( -0.000000000000000000, -1.000000000000000000, -0.000000000000000000 ) ) ;
#48795=PLANE ( 'NONE',  #12773 ) ;
#48796=ADVANCED_FACE ( 'NONE', ( #33506 ), #77791, .T. ) ;
#48797=AXIS2_PLACEMENT_3D ( 'NONE', #94942, #93650, #24260 ) ;
#48798=AXIS2_PLACEMENT_3D ( 'NONE', #73553, #72925, #102394 ) ;
#48799=VERTEX_POINT ( 'NONE', #92398 ) ;
#48800=ORIENTED_EDGE ( 'NONE', *, *, #54720, .T. ) ;
#48801=ORIENTED_EDGE ( 'NONE', *, *, #65340, .F. ) ;
#48802=ORIENTED_EDGE ( 'NONE', *, *, #64024, .T. ) ;
#48803=CONICAL_SURFACE ( 'NONE', #59181, 0.09999999999999982514, 0.003490658503988666988 ) ;
#48804=VERTEX_POINT ( 'NONE', #2726 ) ;
#48805=DIRECTION ( 'NONE',  ( 0.000000000000000000, 1.000000000000000000, 0.000000000000000000 ) ) ;
#48806=CIRCLE ( 'NONE', #52998, 0.06509327318403743123 ) ;
#48808=CARTESIAN_POINT ( 'NONE',  ( -6.050000000000017586, 12.50000000000000000, 1.818653347947321475 ) ) ;
#48809=VERTEX_POINT ( 'NONE', #113987 ) ;
#48810=FACE_BOUND ( 'NONE', #71192, .T. ) ;
#48811=EDGE_CURVE ( 'NONE', #22835, #54447, #120843, .T. ) ;
#48812=CONICAL_SURFACE ( 'NONE', #65508, 0.09999999999999999167, 0.003490658503988666988 ) ;
#48813=DIRECTION ( 'NONE',  ( -0.000000000000000000, 1.000000000000000000, -0.000000000000000000 ) ) ;
#48815=CARTESIAN_POINT ( 'NONE',  ( -5.600000000000020073, 2.500000000000000000, 4.676537180435972552 ) ) ;
#48816=CARTESIAN_POINT ( 'NONE',  ( -8.550000000000013145, 12.50000000000000000, 2.511473670974873507 ) ) ;
#48817=FACE_OUTER_BOUND ( 'NONE', #58595, .T. ) ;
#48818=EDGE_CURVE ( 'NONE', #2356, #55110, #22399, .T. ) ;
#48819=DIRECTION ( 'NONE',  ( -0.000000000000000000, 1.000000000000000000, -0.000000000000000000 ) ) ;
#48820=ORIENTED_EDGE ( 'NONE', *, *, #79864, .F. ) ;
#48821=CIRCLE ( 'NONE', #103090, 0.06509327318403745899 ) ;
#48822=EDGE_LOOP ( 'NONE', ( #85954, #112178 ) ) ;
#48823=ORIENTED_EDGE ( 'NONE', *, *, #70989, .T. ) ;
#48824=ORIENTED_EDGE ( 'NONE', *, *, #79617, .T. ) ;
#48825=DIRECTION ( 'NONE',  ( -0.000000000000000000, 1.000000000000000000, -0.000000000000000000 ) ) ;
#48826=DIRECTION ( 'NONE',  ( 0.000000000000000000, 0.000000000000000000, 1.000000000000000000 ) ) ;
#48827=FACE_OUTER_BOUND ( 'NONE', #114557, .T. ) ;
#48828=ORIENTED_EDGE ( 'NONE', *, *, #118762, .T. ) ;
#48829=DIRECTION ( 'NONE',  ( 0.000000000000000000, -0.9999939076577903929, 0.003490651415223739937 ) ) ;
#48830=AXIS2_PLACEMENT_3D ( 'NONE', #111856, #102031, #91562 ) ;
#48831=AXIS2_PLACEMENT_3D ( 'NONE', #68902, #28349, #78089 ) ;
#48832=AXIS2_PLACEMENT_3D ( 'NONE', #44236, #35720, #75002 ) ;
#48833=DIRECTION ( 'NONE',  ( 0.000000000000000000, 0.000000000000000000, -1.000000000000000000 ) ) ;
#48834=FACE_OUTER_BOUND ( 'NONE', #17881, .T. ) ;
#48836=DIRECTION ( 'NONE',  ( -0.000000000000000000, 1.000000000000000000, -0.000000000000000000 ) ) ;
#48837=DIRECTION ( 'NONE',  ( 0.000000000000000000, -0.000000000000000000, 1.000000000000000000 ) ) ;
#48840=EDGE_LOOP ( 'NONE', ( #61032, #82386 ) ) ;
#48841=PLANE ( 'NONE',  #23273 ) ;
#48842=AXIS2_PLACEMENT_3D ( 'NONE', #19345, #117530, #27238 ) ;
#48843=VERTEX_POINT ( 'NONE', #41393 ) ;
#48844=CIRCLE ( 'NONE', #111520, 0.06509327318403745899 ) ;
#48845=ADVANCED_FACE ( 'NONE', ( #112700 ), #118784, .T. ) ;
#48846=ORIENTED_EDGE ( 'NONE', *, *, #109065, .T. ) ;
#48847=CARTESIAN_POINT ( 'NONE',  ( 8.349999999999919709, 2.500000000000000000, -2.265063509461101798 ) ) ;
#48848=DIRECTION ( 'NONE',  ( -4.274815082592931898E-19, -0.9999939076577903929, -0.003490651415223739937 ) ) ;
#48849=CARTESIAN_POINT ( 'NONE',  ( -5.650000000000019895, 12.50000000000000000, 6.213873640053558134 ) ) ;
#48850=CIRCLE ( 'NONE', #117764, 0.06509327318403745899 ) ;
#48851=EDGE_LOOP ( 'NONE', ( #87304, #83927 ) ) ;
#48852=ORIENTED_EDGE ( 'NONE', *, *, #56596, .F. ) ;
#48853=EDGE_CURVE ( 'NONE', #110877, #127992, #45646, .T. ) ;
#48854=DIRECTION ( 'NONE',  ( -0.000000000000000000, 1.000000000000000000, -0.000000000000000000 ) ) ;
#48856=AXIS2_PLACEMENT_3D ( 'NONE', #122651, #11404, #82747 ) ;
#48857=AXIS2_PLACEMENT_3D ( 'NONE', #78599, #118490, #20303 ) ;
#48858=AXIS2_PLACEMENT_3D ( 'NONE', #49501, #8891, #106459 ) ;
#48859=ORIENTED_EDGE ( 'NONE', *, *, #1396, .F. ) ;
#48860=ORIENTED_EDGE ( 'NONE', *, *, #35840, .F. ) ;
#48861=EDGE_CURVE ( 'NONE', #22448, #33469, #112544, .T. ) ;
#48862=DIRECTION ( 'NONE',  ( -0.000000000000000000, 1.000000000000000000, -0.000000000000000000 ) ) ;
#48863=ADVANCED_FACE ( 'NONE', ( #103523 ), #83865, .T. ) ;
#48864=EDGE_CURVE ( 'NONE', #73617, #58840, #100013, .T. ) ;
#48865=ORIENTED_EDGE ( 'NONE', *, *, #59941, .T. ) ;
#48866=AXIS2_PLACEMENT_3D ( 'NONE', #35585, #75484, #124606 ) ;
#48867=CARTESIAN_POINT ( 'NONE',  ( -6.850000000000013856, 2.500000000000000000, 1.818653347947321475 ) ) ;
#48868=VERTEX_POINT ( 'NONE', #74057 ) ;
#48869=DIRECTION ( 'NONE',  ( 0.000000000000000000, 0.000000000000000000, 1.000000000000000000 ) ) ;
#48870=EDGE_CURVE ( 'NONE', #55120, #32820, #12544, .T. ) ;
#48871=CARTESIAN_POINT ( 'NONE',  ( 6.849999999999927702, 2.500000000000000000, 2.611473670974873151 ) ) ;
#48872=DIRECTION ( 'NONE',  ( 0.000000000000000000, 0.000000000000000000, 1.000000000000000000 ) ) ;
#48873=CARTESIAN_POINT ( 'NONE',  ( -6.250000000000015987, 12.50000000000000000, 1.537336459617582918 ) ) ;
#48874=ORIENTED_EDGE ( 'NONE', *, *, #15968, .T. ) ;
#48875=EDGE_CURVE ( 'NONE', #91777, #32532, #53769, .T. ) ;
#48876=DIRECTION ( 'NONE',  ( -4.274815082592931898E-19, -0.9999939076577903929, -0.003490651415223739937 ) ) ;
#48877=ADVANCED_FACE ( 'NONE', ( #82601 ), #32223, .T. ) ;
#48878=VERTEX_POINT ( 'NONE', #93697 ) ;
#48879=EDGE_LOOP ( 'NONE', ( #53080, #5807, #20091, #106966 ) ) ;
#48880=VECTOR ( 'NONE', #47575, 1000.000000000000000 ) ;
#48881=AXIS2_PLACEMENT_3D ( 'NONE', #61534, #102713, #32080 ) ;
#48882=CARTESIAN_POINT ( 'NONE',  ( -4.150000000000025224, 2.500000000000000000, 6.595190528383296780 ) ) ;
#48883=DIRECTION ( 'NONE',  ( -4.274815082592931898E-19, -0.9999939076577903929, -0.003490651415223739937 ) ) ;
#48884=CARTESIAN_POINT ( 'NONE',  ( 7.899999999999921307, 2.500000000000000000, -2.385244779468109755E-15 ) ) ;
#48885=CARTESIAN_POINT ( 'NONE',  ( 2.499999999999945377, 2.500000000000000000, 5.022947341949748790 ) ) ;
#48886=CARTESIAN_POINT ( 'NONE',  ( 7.099999999999926814, 12.50000000000000000, -0.7579135962115916003 ) ) ;
#48887=DIRECTION ( 'NONE',  ( 0.000000000000000000, 1.000000000000000000, 0.000000000000000000 ) ) ;
#48888=CONICAL_SURFACE ( 'NONE', #128302, 0.1000000000000002554, 0.003490658503988666988 ) ;
#48889=AXIS2_PLACEMENT_3D ( 'NONE', #83649, #60932, #103291 ) ;
#48890=PLANE ( 'NONE',  #67730 ) ;
#48891=AXIS2_PLACEMENT_3D ( 'NONE', #36576, #77127, #7720 ) ;
#48892=FACE_OUTER_BOUND ( 'NONE', #63112, .T. ) ;
#48893=CARTESIAN_POINT ( 'NONE',  ( -7.900000000000014566, 2.500000000000000000, -2.276824562219559311E-15 ) ) ;
#48894=AXIS2_PLACEMENT_3D ( 'NONE', #104521, #54771, #115622 ) ;
#48895=CONICAL_SURFACE ( 'NONE', #73702, 0.1000000000000002554, 0.003490658503988666988 ) ;
#48896=CONICAL_SURFACE ( 'NONE', #55144, 0.1000000000000002554, 0.003490658503988666988 ) ;
#48897=AXIS2_PLACEMENT_3D ( 'NONE', #122571, #91170, #32921 ) ;
#48898=EDGE_LOOP ( 'NONE', ( #47111, #19356, #79780, #42819 ) ) ;
#48899=CARTESIAN_POINT ( 'NONE',  ( 9.799999999999918998, 2.500000000000000000, -0.3464101615137782364 ) ) ;
#48900=CONICAL_SURFACE ( 'NONE', #113634, 0.09999999999999999167, 0.003490658503988666988 ) ;
#48901=DIRECTION ( 'NONE',  ( -0.000000000000000000, 1.000000000000000000, -0.000000000000000000 ) ) ;
#48902=CARTESIAN_POINT ( 'NONE',  ( -5.400000000000019895, 12.50000000000000000, -0.6277270498435166823 ) ) ;
#48903=DIRECTION ( 'NONE',  ( 0.000000000000000000, 0.000000000000000000, 1.000000000000000000 ) ) ;
#48904=CARTESIAN_POINT ( 'NONE',  ( -0.6500000000000398792, 2.500000000000000000, -6.841600689897078702 ) ) ;
#48905=VERTEX_POINT ( 'NONE', #81929 ) ;
#48906=FACE_OUTER_BOUND ( 'NONE', #111680, .T. ) ;
#48907=CARTESIAN_POINT ( 'NONE',  ( 4.399999999999940847, 2.500000000000000000, -3.883716857408426648 ) ) ;
#48908=DIRECTION ( 'NONE',  ( -0.000000000000000000, 1.000000000000000000, -0.000000000000000000 ) ) ;
#48909=ORIENTED_EDGE ( 'NONE', *, *, #1955, .T. ) ;
#48910=AXIS2_PLACEMENT_3D ( 'NONE', #20426, #60374, #100277 ) ;
#48911=ORIENTED_EDGE ( 'NONE', *, *, #114820, .T. ) ;
#48912=CARTESIAN_POINT ( 'NONE',  ( 2.299999999999948752, 2.500000000000000000, -3.983716857408426293 ) ) ;
#48913=EDGE_CURVE ( 'NONE', #59940, #69598, #104161, .T. ) ;
#48915=EDGE_LOOP ( 'NONE', ( #127908, #1045 ) ) ;
#48916=ORIENTED_EDGE ( 'NONE', *, *, #26500, .T. ) ;
#48917=FACE_OUTER_BOUND ( 'NONE', #99375, .T. ) ;
#48918=DIRECTION ( 'NONE',  ( 0.000000000000000000, 0.000000000000000000, 1.000000000000000000 ) ) ;
#48919=CARTESIAN_POINT ( 'NONE',  ( 0.7999999999999612976, 12.50000000000000000, -1.084202172485504434E-16 ) ) ;
#48920=CIRCLE ( 'NONE', #113762, 0.06509327318403745899 ) ;
#48921=LINE ( 'NONE', #108460, #29117 ) ;
#48922=AXIS2_PLACEMENT_3D ( 'NONE', #94974, #125693, #15082 ) ;
#48923=EDGE_LOOP ( 'NONE', ( #4637, #53296, #15405, #113166 ) ) ;
#48924=DIRECTION ( 'NONE',  ( 0.000000000000000000, 1.000000000000000000, 0.000000000000000000 ) ) ;
#48925=ORIENTED_EDGE ( 'NONE', *, *, #95877, .T. ) ;
#48926=DIRECTION ( 'NONE',  ( 0.000000000000000000, 0.000000000000000000, -1.000000000000000000 ) ) ;
#48927=CARTESIAN_POINT ( 'NONE',  ( 15.24415751722251144, -2.474878586409045678, -4.460068884085897523 ) ) ;
#48928=CARTESIAN_POINT ( 'NONE',  ( 15.44463772192102269, 2.469073678227445168, 4.264595835262002588 ) ) ;
#48929=CARTESIAN_POINT ( 'NONE',  ( 10.84999999999991260, 2.500000000000000000, -2.165063509461101710 ) ) ;
#48930=DIRECTION ( 'NONE',  ( -0.000000000000000000, -1.000000000000000000, -0.000000000000000000 ) ) ;
#48931=EDGE_LOOP ( 'NONE', ( #108214, #35921 ) ) ;
#48932=EDGE_LOOP ( 'NONE', ( #106326, #66606, #96085, #74787 ) ) ;
#48933=ORIENTED_EDGE ( 'NONE', *, *, #102290, .F. ) ;
#48934=ORIENTED_EDGE ( 'NONE', *, *, #34044, .F. ) ;
#48935=ORIENTED_EDGE ( 'NONE', *, *, #103221, .F. ) ;
#48936=DIRECTION ( 'NONE',  ( -0.000000000000000000, -1.000000000000000000, -0.000000000000000000 ) ) ;
#48937=CARTESIAN_POINT ( 'NONE',  ( 10.19999999999991225, 2.500000000000000000, -4.676537180435978769 ) ) ;
#48938=DIRECTION ( 'NONE',  ( 0.000000000000000000, 1.000000000000000000, 0.000000000000000000 ) ) ;
#48939=FACE_BOUND ( 'NONE', #9573, .T. ) ;
#48940=DIRECTION ( 'NONE',  ( 0.000000000000000000, 0.000000000000000000, 1.000000000000000000 ) ) ;
#48942=FACE_OUTER_BOUND ( 'NONE', #17064, .T. ) ;
#48943=FACE_OUTER_BOUND ( 'NONE', #103145, .T. ) ;
#48944=AXIS2_PLACEMENT_3D ( 'NONE', #97693, #47968, #87859 ) ;
#48945=AXIS2_PLACEMENT_3D ( 'NONE', #11107, #21591, #39095 ) ;
#48946=CIRCLE ( 'NONE', #23904, 0.06509327318403743123 ) ;
#48947=CARTESIAN_POINT ( 'NONE',  ( 11.84999999999990372, 2.500000000000000000, 2.511473670974873507 ) ) ;
#48948=CARTESIAN_POINT ( 'NONE',  ( -2.950000000000033484, 2.500000000000000000, -6.595190528383302109 ) ) ;
#48949=AXIS2_PLACEMENT_3D ( 'NONE', #95801, #45426, #63777 ) ;
#48950=DIRECTION ( 'NONE',  ( 0.000000000000000000, 0.000000000000000000, 1.000000000000000000 ) ) ;
#48951=CONICAL_SURFACE ( 'NONE', #908, 0.1000000000000000056, 0.003490658503988666988 ) ;
#48952=EDGE_CURVE ( 'NONE', #91341, #69398, #37235, .T. ) ;
#48953=DIRECTION ( 'NONE',  ( 0.000000000000000000, 1.000000000000000000, 0.000000000000000000 ) ) ;
#48954=ORIENTED_EDGE ( 'NONE', *, *, #34308, .T. ) ;
#48955=ORIENTED_EDGE ( 'NONE', *, *, #115752, .F. ) ;
#48956=EDGE_LOOP ( 'NONE', ( #76868, #24181 ) ) ;
#48958=DIRECTION ( 'NONE',  ( 0.000000000000000000, 0.000000000000000000, -1.000000000000000000 ) ) ;
#48959=EDGE_CURVE ( 'NONE', #64702, #16084, #97848, .T. ) ;
#48960=CARTESIAN_POINT ( 'NONE',  ( -3.150000000000030553, 2.500000000000000000, 6.048780366869520364 ) ) ;
#48961=FACE_BOUND ( 'NONE', #85376, .T. ) ;
#48962=EDGE_CURVE ( 'NONE', #68417, #66442, #107219, .T. ) ;
#48963=CARTESIAN_POINT ( 'NONE',  ( -11.89999999999999503, 2.500000000000000000, 3.983716857408420076 ) ) ;
#48964=ADVANCED_FACE ( 'NONE', ( #87570 ), #28921, .T. ) ;
#48965=VECTOR ( 'NONE', #77043, 1000.000000000000000 ) ;
#48966=ADVANCED_FACE ( 'NONE', ( #79068 ), #102070, .T. ) ;
#48967=AXIS2_PLACEMENT_3D ( 'NONE', #19373, #27923, #59344 ) ;
#48968=VERTEX_POINT ( 'NONE', #78436 ) ;
#48969=DIRECTION ( 'NONE',  ( 0.000000000000000000, 0.000000000000000000, 1.000000000000000000 ) ) ;
#48970=AXIS2_PLACEMENT_3D ( 'NONE', #101301, #71842, #29987 ) ;
#48971=LINE ( 'NONE', #88875, #53578 ) ;
#48972=DIRECTION ( 'NONE',  ( 0.000000000000000000, 0.000000000000000000, 1.000000000000000000 ) ) ;
#48973=EDGE_CURVE ( 'NONE', #68081, #20474, #47695, .T. ) ;
#48974=DIRECTION ( 'NONE',  ( 0.000000000000000000, 0.000000000000000000, 1.000000000000000000 ) ) ;
#48975=ORIENTED_EDGE ( 'NONE', *, *, #3901, .F. ) ;
#48976=CARTESIAN_POINT ( 'NONE',  ( 3.149999999999946176, 12.50000000000000000, -6.148780366869526226 ) ) ;
#48977=CIRCLE ( 'NONE', #13444, 0.1000000000000002554 ) ;
#48978=AXIS2_PLACEMENT_3D ( 'NONE', #4256, #114866, #13445 ) ;
#48979=CIRCLE ( 'NONE', #126232, 0.09999999999999982514 ) ;
#48980=AXIS2_PLACEMENT_3D ( 'NONE', #97614, #124668, #7936 ) ;
#48981=EDGE_LOOP ( 'NONE', ( #16233, #68716 ) ) ;
#48982=ORIENTED_EDGE ( 'NONE', *, *, #5112, .F. ) ;
#48983=DIRECTION ( 'NONE',  ( -0.000000000000000000, -1.000000000000000000, -0.000000000000000000 ) ) ;
#48984=DIRECTION ( 'NONE',  ( 0.000000000000000000, 0.000000000000000000, -1.000000000000000000 ) ) ;
#48985=EDGE_LOOP ( 'NONE', ( #107616, #86160, #123154, #36793 ) ) ;
#48986=CONICAL_SURFACE ( 'NONE', #46930, 0.09999999999999982514, 0.003490658503988666988 ) ;
#48987=VECTOR ( 'NONE', #22163, 1000.000000000000000 ) ;
#48988=AXIS2_PLACEMENT_3D ( 'NONE', #17861, #78749, #118640 ) ;
#48989=DIRECTION ( 'NONE',  ( 0.000000000000000000, 1.000000000000000000, 0.000000000000000000 ) ) ;
#48990=FACE_OUTER_BOUND ( 'NONE', #41688, .T. ) ;
#48991=VERTEX_POINT ( 'NONE', #118975 ) ;
#48992=DIRECTION ( 'NONE',  ( 0.000000000000000000, 0.000000000000000000, 1.000000000000000000 ) ) ;
#48993=CONICAL_SURFACE ( 'NONE', #46940, 0.09999999999999999167, 0.003490658503988666988 ) ;
#48994=EDGE_LOOP ( 'NONE', ( #7965, #48802, #94307, #27443 ) ) ;
#48995=DIRECTION ( 'NONE',  ( 0.000000000000000000, 0.000000000000000000, 1.000000000000000000 ) ) ;
#48996=ORIENTED_EDGE ( 'NONE', *, *, #49037, .F. ) ;
#48997=PLANE ( 'NONE',  #51319 ) ;
#48998=FACE_BOUND ( 'NONE', #5620, .T. ) ;
#48999=ORIENTED_EDGE ( 'NONE', *, *, #91798, .F. ) ;
#49001=ORIENTED_EDGE ( 'NONE', *, *, #85274, .T. ) ;
#49002=CARTESIAN_POINT ( 'NONE',  ( -5.650000000000023448, 2.500000000000000000, -2.611473670974877592 ) ) ;
#49003=DIRECTION ( 'NONE',  ( 0.000000000000000000, 0.000000000000000000, 1.000000000000000000 ) ) ;
#49004=CARTESIAN_POINT ( 'NONE',  ( 2.699999999999947331, 12.50000000000000000, -4.676537180435978769 ) ) ;
#49005=FACE_OUTER_BOUND ( 'NONE', #35710, .T. ) ;
#49006=DIRECTION ( 'NONE',  ( 0.000000000000000000, 0.000000000000000000, 1.000000000000000000 ) ) ;
#49007=CIRCLE ( 'NONE', #122162, 0.06509327318403741736 ) ;
#49009=ORIENTED_EDGE ( 'NONE', *, *, #55522, .F. ) ;
#49010=VERTEX_POINT ( 'NONE', #28673 ) ;
#49011=DIRECTION ( 'NONE',  ( -4.274815082592931898E-19, -0.9999939076577903929, -0.003490651415223739937 ) ) ;
#49012=DIRECTION ( 'NONE',  ( 0.000000000000000000, -0.000000000000000000, 1.000000000000000000 ) ) ;
#49013=CARTESIAN_POINT ( 'NONE',  ( 4.599999999999940137, 12.50000000000000000, -5.022947341949754119 ) ) ;
#49014=EDGE_CURVE ( 'NONE', #24765, #27897, #64405, .T. ) ;
#49015=VERTEX_POINT ( 'NONE', #69217 ) ;
#49016=EDGE_LOOP ( 'NONE', ( #30052, #83094 ) ) ;
#49017=ORIENTED_EDGE ( 'NONE', *, *, #100064, .F. ) ;
#49018=EDGE_CURVE ( 'NONE', #109103, #73593, #37836, .T. ) ;
#49019=PLANE ( 'NONE',  #83330 ) ;
#49020=EDGE_CURVE ( 'NONE', #29970, #128096, #86274, .T. ) ;
#49021=AXIS2_PLACEMENT_3D ( 'NONE', #18689, #69076, #60580 ) ;
#49022=FACE_OUTER_BOUND ( 'NONE', #47069, .T. ) ;
#49023=AXIS2_PLACEMENT_3D ( 'NONE', #53609, #63424, #71968 ) ;
#49024=CARTESIAN_POINT ( 'NONE',  ( 8.349999999999919709, 2.500000000000000000, -2.165063509461101710 ) ) ;
#49025=DIRECTION ( 'NONE',  ( 0.000000000000000000, 1.000000000000000000, 0.000000000000000000 ) ) ;
#49026=DIRECTION ( 'NONE',  ( 0.000000000000000000, 1.000000000000000000, 0.000000000000000000 ) ) ;
#49027=CARTESIAN_POINT ( 'NONE',  ( -4.400000000000028777, 12.50000000000000000, -4.676537180435978769 ) ) ;
#49028=CARTESIAN_POINT ( 'NONE',  ( -11.25000000000000178, 12.50000000000000000, -5.737276932171709198 ) ) ;
#49029=EDGE_CURVE ( 'NONE', #123681, #57299, #3859, .T. ) ;
#49031=DIRECTION ( 'NONE',  ( 0.000000000000000000, -0.9999939076577903929, 0.003490651415223739937 ) ) ;
#49032=EDGE_CURVE ( 'NONE', #50883, #108236, #77023, .T. ) ;
#49034=EDGE_CURVE ( 'NONE', #18830, #93842, #93755, .T. ) ;
#49035=ORIENTED_EDGE ( 'NONE', *, *, #17925, .F. ) ;
#49036=DIRECTION ( 'NONE',  ( 0.000000000000000000, 0.000000000000000000, 1.000000000000000000 ) ) ;
#49037=EDGE_CURVE ( 'NONE', #63511, #53411, #22658, .T. ) ;
#49038=CARTESIAN_POINT ( 'NONE',  ( 4.149999999999936406, 2.500000000000000000, 6.395190528383296602 ) ) ;
#49039=ORIENTED_EDGE ( 'NONE', *, *, #16327, .T. ) ;
#49040=ORIENTED_EDGE ( 'NONE', *, *, #73994, .T. ) ;
#49042=DIRECTION ( 'NONE',  ( 0.000000000000000000, 0.000000000000000000, -1.000000000000000000 ) ) ;
#49043=DIRECTION ( 'NONE',  ( 0.000000000000000000, 0.000000000000000000, 1.000000000000000000 ) ) ;
#49044=ADVANCED_FACE ( 'NONE', ( #68579 ), #18440, .T. ) ;
#49045=LINE ( 'NONE', #79146, #121500 ) ;
#49046=CIRCLE ( 'NONE', #61558, 0.09999999999999982514 ) ;
#49048=AXIS2_PLACEMENT_3D ( 'NONE', #115584, #14787, #35133 ) ;
#49049=LINE ( 'NONE', #69964, #26003 ) ;
#49050=DIRECTION ( 'NONE',  ( 0.000000000000000000, 1.000000000000000000, 0.000000000000000000 ) ) ;
#49051=CIRCLE ( 'NONE', #17623, 0.1000000000000000472 ) ;
#49052=CIRCLE ( 'NONE', #72115, 0.1000000000000000472 ) ;
#49053=CARTESIAN_POINT ( 'NONE',  ( -4.800000000000024691, 2.500000000000000000, 0.3464101615137735735 ) ) ;
#49054=VERTEX_POINT ( 'NONE', #47031 ) ;
#49055=ORIENTED_EDGE ( 'NONE', *, *, #9016, .F. ) ;
#49056=VERTEX_POINT ( 'NONE', #47670 ) ;
#49057=ORIENTED_EDGE ( 'NONE', *, *, #63482, .F. ) ;
#49058=CARTESIAN_POINT ( 'NONE',  ( -8.150000000000012790, 2.500000000000000000, -1.718653347947326049 ) ) ;
#49059=LINE ( 'NONE', #129565, #79147 ) ;
#49060=EDGE_LOOP ( 'NONE', ( #80388, #42594, #104913, #9331 ) ) ;
#49061=DIRECTION ( 'NONE',  ( 0.000000000000000000, 0.000000000000000000, 1.000000000000000000 ) ) ;
#49062=CARTESIAN_POINT ( 'NONE',  ( 3.949999999999938005, 2.500000000000000000, 6.841600689897072485 ) ) ;
#49063=CIRCLE ( 'NONE', #122210, 0.1000000000000002554 ) ;
#49064=AXIS2_PLACEMENT_3D ( 'NONE', #42278, #13441, #2321 ) ;
#49065=LINE ( 'NONE', #77849, #118001 ) ;
#49066=LINE ( 'NONE', #109911, #43365 ) ;
#49067=ORIENTED_EDGE ( 'NONE', *, *, #95497, .F. ) ;
#49068=AXIS2_PLACEMENT_3D ( 'NONE', #95230, #55301, #5538 ) ;
#49069=DIRECTION ( 'NONE',  ( 0.000000000000000000, 0.000000000000000000, -1.000000000000000000 ) ) ;
#49070=DIRECTION ( 'NONE',  ( -0.000000000000000000, 1.000000000000000000, -0.000000000000000000 ) ) ;
#49071=VERTEX_POINT ( 'NONE', #48305 ) ;
#49072=AXIS2_PLACEMENT_3D ( 'NONE', #111118, #10992, #70576 ) ;
#49073=EDGE_CURVE ( 'NONE', #28513, #29920, #114568, .T. ) ;
#49074=CIRCLE ( 'NONE', #67828, 0.06509327318403745899 ) ;
#49075=AXIS2_PLACEMENT_3D ( 'NONE', #54513, #112812, #14585 ) ;
#49076=ORIENTED_EDGE ( 'NONE', *, *, #44362, .F. ) ;
#49077=ORIENTED_EDGE ( 'NONE', *, *, #20766, .T. ) ;
#49078=EDGE_LOOP ( 'NONE', ( #1431, #102473 ) ) ;
#49079=DIRECTION ( 'NONE',  ( 0.000000000000000000, 0.000000000000000000, 1.000000000000000000 ) ) ;
#49080=CIRCLE ( 'NONE', #118291, 0.06509327318403741736 ) ;
#49081=DIRECTION ( 'NONE',  ( 0.000000000000000000, -0.9999939076577903929, 0.003490651415223739937 ) ) ;
#49082=CARTESIAN_POINT ( 'NONE',  ( 14.99999999999989164, 2.500000000000000000, 0.6928203230275494784 ) ) ;
#49083=CIRCLE ( 'NONE', #99252, 0.1000000000000002554 ) ;
#49084=AXIS2_PLACEMENT_3D ( 'NONE', #43178, #52979, #83095 ) ;
#49085=AXIS2_PLACEMENT_3D ( 'NONE', #97329, #7644, #95396 ) ;
#49086=EDGE_LOOP ( 'NONE', ( #124160, #14890 ) ) ;
#49087=DIRECTION ( 'NONE',  ( 0.000000000000000000, -0.000000000000000000, -1.000000000000000000 ) ) ;
#49088=DIRECTION ( 'NONE',  ( 0.000000000000000000, -0.000000000000000000, 1.000000000000000000 ) ) ;
#49089=EDGE_CURVE ( 'NONE', #33171, #102865, #18836, .T. ) ;
#49090=CARTESIAN_POINT ( 'NONE',  ( -8.550000000000014921, 2.500000000000000000, -6.248780366869521430 ) ) ;
#49092=VERTEX_POINT ( 'NONE', #58773 ) ;
#49093=DIRECTION ( 'NONE',  ( 0.000000000000000000, 0.000000000000000000, 1.000000000000000000 ) ) ;
#49094=ORIENTED_EDGE ( 'NONE', *, *, #110731, .F. ) ;
#49096=PLANE ( 'NONE',  #16224 ) ;
#49097=DIRECTION ( 'NONE',  ( -0.000000000000000000, 1.000000000000000000, -0.000000000000000000 ) ) ;
#49098=FACE_BOUND ( 'NONE', #79508, .T. ) ;
#49099=DIRECTION ( 'NONE',  ( -4.274815082592931898E-19, -0.9999939076577903929, -0.003490651415223739937 ) ) ;
#49100=CONICAL_SURFACE ( 'NONE', #74133, 0.1000000000000000056, 0.003490658503988666988 ) ;
#49101=DIRECTION ( 'NONE',  ( 0.000000000000000000, 0.000000000000000000, 1.000000000000000000 ) ) ;
#49103=EDGE_LOOP ( 'NONE', ( #35193, #57057, #66304, #36764 ) ) ;
#49104=FACE_OUTER_BOUND ( 'NONE', #85836, .T. ) ;
#49105=DIRECTION ( 'NONE',  ( 0.000000000000000000, 0.000000000000000000, 1.000000000000000000 ) ) ;
#49106=CARTESIAN_POINT ( 'NONE',  ( -12.89999999999999147, 2.500000000000000000, 4.230127018922196669 ) ) ;
#49108=VERTEX_POINT ( 'NONE', #96741 ) ;
#49109=AXIS2_PLACEMENT_3D ( 'NONE', #19323, #68432, #109661 ) ;
#49110=CONICAL_SURFACE ( 'NONE', #59590, 0.1000000000000002554, 0.003490658503988666988 ) ;
#49112=EDGE_CURVE ( 'NONE', #64688, #61872, #7966, .T. ) ;
#49113=FACE_OUTER_BOUND ( 'NONE', #771, .T. ) ;
#49114=VERTEX_POINT ( 'NONE', #1766 ) ;
#49115=ORIENTED_EDGE ( 'NONE', *, *, #123838, .T. ) ;
#49116=DIRECTION ( 'NONE',  ( 0.000000000000000000, 0.000000000000000000, 1.000000000000000000 ) ) ;
#49117=DIRECTION ( 'NONE',  ( 0.000000000000000000, 0.000000000000000000, 1.000000000000000000 ) ) ;
#49118=FACE_BOUND ( 'NONE', #57384, .T. ) ;
#49119=EDGE_CURVE ( 'NONE', #125645, #86214, #108315, .T. ) ;
#49120=CARTESIAN_POINT ( 'NONE',  ( 1.699999999999951994, 2.500000000000000000, -4.330127018922201643 ) ) ;
#49121=CIRCLE ( 'NONE', #82566, 0.1000000000000002554 ) ;
#49122=VERTEX_POINT ( 'NONE', #70514 ) ;
#49123=FACE_OUTER_BOUND ( 'NONE', #92791, .T. ) ;
#49124=CIRCLE ( 'NONE', #59602, 0.06509327318403745899 ) ;
#49125=ADVANCED_FACE ( 'NONE', ( #20783 ), #72829, .T. ) ;
#49127=ORIENTED_EDGE ( 'NONE', *, *, #124788, .F. ) ;
#49128=CARTESIAN_POINT ( 'NONE',  ( 12.09999999999990550, 2.500000000000000000, 3.537306695894645081 ) ) ;
#49129=ADVANCED_FACE ( 'NONE', ( #50886 ), #129378, .T. ) ;
#49130=ADVANCED_FACE ( 'NONE', ( #99349 ), #24797, .T. ) ;
#49132=ADVANCED_FACE ( 'NONE', ( #71819 ), #2400, .T. ) ;
#49133=EDGE_LOOP ( 'NONE', ( #122299, #105879 ) ) ;
#49134=DIRECTION ( 'NONE',  ( 0.000000000000000000, 0.000000000000000000, 1.000000000000000000 ) ) ;
#49136=AXIS2_PLACEMENT_3D ( 'NONE', #57631, #99494, #9813 ) ;
#49137=AXIS2_PLACEMENT_3D ( 'NONE', #89996, #99846, #316 ) ;
#49138=DIRECTION ( 'NONE',  ( 0.000000000000000000, 1.000000000000000000, 0.000000000000000000 ) ) ;
#49139=FACE_OUTER_BOUND ( 'NONE', #108080, .T. ) ;
#49140=ADVANCED_FACE ( 'NONE', ( #82286 ), #129474, .T. ) ;
#49141=EDGE_CURVE ( 'NONE', #66521, #107226, #50248, .T. ) ;
#49142=ADVANCED_FACE ( 'NONE', ( #122209 ), #60413, .T. ) ;
#49143=EDGE_LOOP ( 'NONE', ( #153, #31503, #36017, #68767 ) ) ;
#49144=CARTESIAN_POINT ( 'NONE',  ( 2.899999999999946620, 12.50000000000000000, -5.022947341949754119 ) ) ;
#49145=CARTESIAN_POINT ( 'NONE',  ( 0.6499999999999561684, 2.500000000000000000, -1.918653347947325782 ) ) ;
#49146=CARTESIAN_POINT ( 'NONE',  ( 13.74999999999989697, 2.500000000000000000, 2.757883832488649656 ) ) ;
#49147=DIRECTION ( 'NONE',  ( -4.274815082592931898E-19, -0.9999939076577903929, -0.003490651415223739937 ) ) ;
#49148=ORIENTED_EDGE ( 'NONE', *, *, #119846, .F. ) ;
#49149=VERTEX_POINT ( 'NONE', #60712 ) ;
#49150=CARTESIAN_POINT ( 'NONE',  ( 15.83209681635555377, 2.500000000000000000, 5.404881881984148428 ) ) ;
#49151=AXIS2_PLACEMENT_3D ( 'NONE', #115135, #25484, #34034 ) ;
#49152=ORIENTED_EDGE ( 'NONE', *, *, #20185, .T. ) ;
#49153=CARTESIAN_POINT ( 'NONE',  ( -7.900000000000014566, 12.50000000000000000, -2.276824562219559311E-15 ) ) ;
#49154=DIRECTION ( 'NONE',  ( -0.000000000000000000, -1.000000000000000000, -0.000000000000000000 ) ) ;
#49155=CARTESIAN_POINT ( 'NONE',  ( -9.150000000000005684, 2.500000000000000000, 7.088010851410848190 ) ) ;
#49156=AXIS2_PLACEMENT_3D ( 'NONE', #58223, #107941, #66077 ) ;
#49157=CARTESIAN_POINT ( 'NONE',  ( -1.050000000000037792, 2.500000000000000000, 6.048780366869520364 ) ) ;
#49158=ORIENTED_EDGE ( 'NONE', *, *, #21934, .T. ) ;
#49159=CONICAL_SURFACE ( 'NONE', #61767, 0.1000000000000002554, 0.003490658503988666988 ) ;
#49160=CARTESIAN_POINT ( 'NONE',  ( 13.34999999999990017, 2.500000000000000000, 2.065063509461097624 ) ) ;
#49161=LINE ( 'NONE', #119164, #66877 ) ;
#49162=CARTESIAN_POINT ( 'NONE',  ( 5.849999999999933920, 12.50000000000000000, 6.495190528383297135 ) ) ;
#49163=AXIS2_PLACEMENT_3D ( 'NONE', #38, #20334, #19690 ) ;
#49165=DIRECTION ( 'NONE',  ( 0.000000000000000000, -0.9999939076577903929, 0.003490651415223739937 ) ) ;
#49166=PLANE ( 'NONE',  #66217 ) ;
#49167=ORIENTED_EDGE ( 'NONE', *, *, #2846, .F. ) ;
#49168=VECTOR ( 'NONE', #44463, 1000.000000000000000 ) ;
#49169=ORIENTED_EDGE ( 'NONE', *, *, #63007, .T. ) ;
#49170=CONICAL_SURFACE ( 'NONE', #57472, 0.09999999999999999167, 0.003490658503988666988 ) ;
#49171=CARTESIAN_POINT ( 'NONE',  ( -5.850000000000022737, 12.50000000000000000, -6.495190528383302464 ) ) ;
#49172=ORIENTED_EDGE ( 'NONE', *, *, #46927, .F. ) ;
#49174=AXIS2_PLACEMENT_3D ( 'NONE', #62746, #55493, #53561 ) ;
#49175=EDGE_LOOP ( 'NONE', ( #81360, #96452 ) ) ;
#49176=EDGE_LOOP ( 'NONE', ( #111303, #61206 ) ) ;
#49177=ORIENTED_EDGE ( 'NONE', *, *, #108373, .F. ) ;
#49178=DIRECTION ( 'NONE',  ( 0.000000000000000000, -0.000000000000000000, 1.000000000000000000 ) ) ;
#49179=EDGE_CURVE ( 'NONE', #64508, #87351, #33223, .T. ) ;
#49180=AXIS2_PLACEMENT_3D ( 'NONE', #44860, #83498, #112942 ) ;
#49182=CIRCLE ( 'NONE', #57478, 0.06509327318403745899 ) ;
#49183=DIRECTION ( 'NONE',  ( -0.000000000000000000, -1.000000000000000000, -0.000000000000000000 ) ) ;
#49184=ADVANCED_FACE ( 'NONE', ( #29965 ), #102160, .T. ) ;
#49185=DIRECTION ( 'NONE',  ( 0.000000000000000000, 0.000000000000000000, 1.000000000000000000 ) ) ;
#49186=DIRECTION ( 'NONE',  ( -0.000000000000000000, 1.000000000000000000, -0.000000000000000000 ) ) ;
#49187=AXIS2_PLACEMENT_3D ( 'NONE', #395, #11523, #90733 ) ;
#49188=DIRECTION ( 'NONE',  ( -4.274815082592931898E-19, -0.9999939076577903929, -0.003490651415223739937 ) ) ;
#49189=DIRECTION ( 'NONE',  ( 0.000000000000000000, 0.000000000000000000, 1.000000000000000000 ) ) ;
#49190=ADVANCED_FACE ( 'NONE', ( #19479 ), #41540, .T. ) ;
#49191=CARTESIAN_POINT ( 'NONE',  ( -10.00000000000000533, 12.50000000000000000, -5.022947341949749678 ) ) ;
#49192=EDGE_LOOP ( 'NONE', ( #2861, #35322 ) ) ;
#49193=ADVANCED_FACE ( 'NONE', ( #101269 ), #41089, .T. ) ;
#49195=EDGE_CURVE ( 'NONE', #64554, #43896, #120905, .T. ) ;
#49196=DIRECTION ( 'NONE',  ( 0.000000000000000000, 0.000000000000000000, 1.000000000000000000 ) ) ;
#49197=ORIENTED_EDGE ( 'NONE', *, *, #73347, .T. ) ;
#49198=EDGE_LOOP ( 'NONE', ( #27794, #5107, #98809, #18739 ) ) ;
#49199=DIRECTION ( 'NONE',  ( -4.274815082592931898E-19, -0.9999939076577903929, -0.003490651415223739937 ) ) ;
#49200=AXIS2_PLACEMENT_3D ( 'NONE', #75503, #38173, #76169 ) ;
#49201=EDGE_CURVE ( 'NONE', #27399, #48060, #109807, .T. ) ;
#49202=DIRECTION ( 'NONE',  ( -4.274815082592931898E-19, -0.9999939076577903929, -0.003490651415223739937 ) ) ;
#49203=PLANE ( 'NONE',  #35893 ) ;
#49204=LINE ( 'NONE', #71373, #95022 ) ;
#49205=DIRECTION ( 'NONE',  ( 0.000000000000000000, -0.9999939076577903929, 0.003490651415223739937 ) ) ;
#49206=ORIENTED_EDGE ( 'NONE', *, *, #27416, .F. ) ;
#49207=AXIS2_PLACEMENT_3D ( 'NONE', #55723, #65542, #115257 ) ;
#49208=AXIS2_PLACEMENT_3D ( 'NONE', #114173, #55255, #104348 ) ;
#49209=VECTOR ( 'NONE', #111721, 1000.000000000000000 ) ;
#49210=VERTEX_POINT ( 'NONE', #21418 ) ;
#49211=DIRECTION ( 'NONE',  ( -0.000000000000000000, 1.000000000000000000, -0.000000000000000000 ) ) ;
#49212=ORIENTED_EDGE ( 'NONE', *, *, #70626, .T. ) ;
#49213=DIRECTION ( 'NONE',  ( 0.000000000000000000, 0.000000000000000000, -1.000000000000000000 ) ) ;
#49215=ADVANCED_FACE ( 'NONE', ( #31894 ), #93841, .T. ) ;
#49217=DIRECTION ( 'NONE',  ( 0.000000000000000000, 1.000000000000000000, 0.000000000000000000 ) ) ;
#49218=LINE ( 'NONE', #70134, #50601 ) ;
#49219=AXIS2_PLACEMENT_3D ( 'NONE', #64840, #13149, #123749 ) ;
#49220=DIRECTION ( 'NONE',  ( -0.000000000000000000, -1.000000000000000000, -0.000000000000000000 ) ) ;
#49221=DIRECTION ( 'NONE',  ( -0.000000000000000000, -1.000000000000000000, -0.000000000000000000 ) ) ;
#49222=CIRCLE ( 'NONE', #111994, 0.06509327318403745899 ) ;
#49223=CARTESIAN_POINT ( 'NONE',  ( -7.950000000000009059, 12.50000000000000000, 6.495190528383297135 ) ) ;
#49224=VERTEX_POINT ( 'NONE', #124126 ) ;
#49225=DIRECTION ( 'NONE',  ( -4.274815082592931898E-19, -0.9999939076577903929, -0.003490651415223739937 ) ) ;
#49226=DIRECTION ( 'NONE',  ( 0.000000000000000000, 0.000000000000000000, -1.000000000000000000 ) ) ;
#49227=CARTESIAN_POINT ( 'NONE',  ( 13.74999999999993427, 2.500000000000000000, 2.065063509461097624 ) ) ;
#49228=LINE ( 'NONE', #28283, #101656 ) ;
#49229=DIRECTION ( 'NONE',  ( -4.274815082592931898E-19, -0.9999939076577903929, -0.003490651415223739937 ) ) ;
#49230=VERTEX_POINT ( 'NONE', #73730 ) ;
#49231=CONICAL_SURFACE ( 'NONE', #107700, 0.1000000000000000472, 0.003490658503988666988 ) ;
#49232=AXIS2_PLACEMENT_3D ( 'NONE', #8067, #37549, #99036 ) ;
#49233=EDGE_CURVE ( 'NONE', #99389, #55154, #29010, .T. ) ;
#49234=EDGE_LOOP ( 'NONE', ( #3816, #5135, #61436, #56946 ) ) ;
#49235=CARTESIAN_POINT ( 'NONE',  ( -1.650000000000034328, 2.500000000000000000, -2.757883832488654097 ) ) ;
#49236=VERTEX_POINT ( 'NONE', #84197 ) ;
#49237=DIRECTION ( 'NONE',  ( 0.000000000000000000, 0.000000000000000000, 1.000000000000000000 ) ) ;
#49238=CARTESIAN_POINT ( 'NONE',  ( 2.499999999999947153, 12.50000000000000000, -3.702399969078687292 ) ) ;
#49239=ORIENTED_EDGE ( 'NONE', *, *, #78258, .F. ) ;
#49240=CARTESIAN_POINT ( 'NONE',  ( 13.34999999999990017, 2.500000000000000000, 2.065063509461097624 ) ) ;
#49241=FACE_OUTER_BOUND ( 'NONE', #48985, .T. ) ;
#49242=EDGE_CURVE ( 'NONE', #10224, #82327, #114941, .T. ) ;
#49243=DIRECTION ( 'NONE',  ( 0.000000000000000000, 1.000000000000000000, 0.000000000000000000 ) ) ;
#49244=VECTOR ( 'NONE', #18251, 1000.000000000000000 ) ;
#49245=DIRECTION ( 'NONE',  ( 0.000000000000000000, 0.000000000000000000, 1.000000000000000000 ) ) ;
#49247=DIRECTION ( 'NONE',  ( 0.000000000000000000, 1.000000000000000000, 0.000000000000000000 ) ) ;
#49248=AXIS2_PLACEMENT_3D ( 'NONE', #94424, #45353, #85262 ) ;
#49249=ORIENTED_EDGE ( 'NONE', *, *, #106971, .T. ) ;
#49250=CARTESIAN_POINT ( 'NONE',  ( 21.23528140090949634, 2.699413673072310171, -2.293764360948883141 ) ) ;
#49251=FACE_OUTER_BOUND ( 'NONE', #56069, .T. ) ;
#49252=CARTESIAN_POINT ( 'NONE',  ( 0.6499999999999566125, 2.500000000000000000, -6.148780366869526226 ) ) ;
#49253=VERTEX_POINT ( 'NONE', #22731 ) ;
#49254=AXIS2_PLACEMENT_3D ( 'NONE', #115986, #54486, #105531 ) ;
#49255=CARTESIAN_POINT ( 'NONE',  ( 1.649999999999950617, 2.500000000000000000, -2.165063509461101710 ) ) ;
#49256=CONICAL_SURFACE ( 'NONE', #59728, 0.1000000000000002554, 0.003490658503988666988 ) ;
#49257=ORIENTED_EDGE ( 'NONE', *, *, #44869, .T. ) ;
#49258=DIRECTION ( 'NONE',  ( 0.000000000000000000, 0.000000000000000000, 1.000000000000000000 ) ) ;
#49259=DIRECTION ( 'NONE',  ( -0.000000000000000000, 1.000000000000000000, -0.000000000000000000 ) ) ;
#49260=DIRECTION ( 'NONE',  ( 0.000000000000000000, 1.000000000000000000, 0.000000000000000000 ) ) ;
#49261=ORIENTED_EDGE ( 'NONE', *, *, #122072, .F. ) ;
#49262=AXIS2_PLACEMENT_3D ( 'NONE', #36968, #38927, #106968 ) ;
#49263=VECTOR ( 'NONE', #99035, 1000.000000000000000 ) ;
#49264=CARTESIAN_POINT ( 'NONE',  ( 7.699999999999923794, 2.500000000000000000, 4.776537180435972196 ) ) ;
#49265=CIRCLE ( 'NONE', #118202, 0.06509327318403745899 ) ;
#49266=ADVANCED_FACE ( 'NONE', ( #73103 ), #44273, .T. ) ;
#49267=LINE ( 'NONE', #117301, #11877 ) ;
#49268=CONICAL_SURFACE ( 'NONE', #74382, 0.1000000000000002554, 0.003490658503988666988 ) ;
#49269=ORIENTED_EDGE ( 'NONE', *, *, #100239, .F. ) ;
#49270=PLANE ( 'NONE',  #34283 ) ;
#49271=ORIENTED_EDGE ( 'NONE', *, *, #89737, .T. ) ;
#49272=LINE ( 'NONE', #79999, #124779 ) ;
#49273=ADVANCED_FACE ( 'NONE', ( #113673 ), #74388, .T. ) ;
#49274=EDGE_LOOP ( 'NONE', ( #46981, #20468, #100656, #14778 ) ) ;
#49275=DIRECTION ( 'NONE',  ( -0.000000000000000000, -1.000000000000000000, -0.000000000000000000 ) ) ;
#49277=ADVANCED_FACE ( 'NONE', ( #14159 ), #85426, .T. ) ;
#49278=ORIENTED_EDGE ( 'NONE', *, *, #112240, .F. ) ;
#49279=ADVANCED_FACE ( 'NONE', ( #102550 ), #14310, .T. ) ;
#49280=ORIENTED_EDGE ( 'NONE', *, *, #120476, .F. ) ;
#49281=EDGE_CURVE ( 'NONE', #67302, #12498, #43693, .T. ) ;
#49282=EDGE_CURVE ( 'NONE', #66379, #55337, #54132, .T. ) ;
#49283=CARTESIAN_POINT ( 'NONE',  ( -1.650000000000035216, 12.50000000000000000, -5.802370205355749988 ) ) ;
#49284=CARTESIAN_POINT ( 'NONE',  ( -3.550000000000030909, 2.500000000000000000, -6.741600689897078169 ) ) ;
#49285=AXIS2_PLACEMENT_3D ( 'NONE', #65535, #7897, #26269 ) ;
#49286=ORIENTED_EDGE ( 'NONE', *, *, #105533, .F. ) ;
#49287=DIRECTION ( 'NONE',  ( 0.000000000000000000, -0.000000000000000000, 1.000000000000000000 ) ) ;
#49288=CARTESIAN_POINT ( 'NONE',  ( -6.900000000000019007, 2.500000000000000000, -3.983716857408426293 ) ) ;
#49289=ADVANCED_FACE ( 'NONE', ( #94025 ), #43029, .T. ) ;
#49291=DIRECTION ( 'NONE',  ( -0.000000000000000000, -1.000000000000000000, -0.000000000000000000 ) ) ;
#49292=ADVANCED_FACE ( 'NONE', ( #3078 ), #108409, .T. ) ;
#49293=CARTESIAN_POINT ( 'NONE',  ( -6.450000000000014388, 2.500000000000000000, 6.048780366869521252 ) ) ;
#49294=AXIS2_PLACEMENT_3D ( 'NONE', #29493, #127683, #97577 ) ;
#49295=DIRECTION ( 'NONE',  ( 0.000000000000000000, 0.000000000000000000, 1.000000000000000000 ) ) ;
#49296=EDGE_CURVE ( 'NONE', #16549, #128756, #5629, .T. ) ;
#49297=AXIS2_PLACEMENT_3D ( 'NONE', #107705, #9505, #18019 ) ;
#49298=EDGE_CURVE ( 'NONE', #66944, #120047, #87472, .T. ) ;
#49299=EDGE_CURVE ( 'NONE', #58340, #93836, #83579, .T. ) ;
#49300=EDGE_LOOP ( 'NONE', ( #44582, #30647, #92229, #80880 ) ) ;
#49301=VECTOR ( 'NONE', #42681, 1000.000000000000000 ) ;
#49302=EDGE_LOOP ( 'NONE', ( #58732, #81418 ) ) ;
#49303=ORIENTED_EDGE ( 'NONE', *, *, #69301, .F. ) ;
#49304=ORIENTED_EDGE ( 'NONE', *, *, #62863, .T. ) ;
#49305=DIRECTION ( 'NONE',  ( -0.000000000000000000, -1.000000000000000000, -0.000000000000000000 ) ) ;
#49306=DIRECTION ( 'NONE',  ( 0.000000000000000000, 0.000000000000000000, -1.000000000000000000 ) ) ;
#49307=CARTESIAN_POINT ( 'NONE',  ( -3.550000000000030909, 2.500000000000000000, -6.841600689897078702 ) ) ;
#49308=ORIENTED_EDGE ( 'NONE', *, *, #67223, .T. ) ;
#49309=FACE_BOUND ( 'NONE', #74299, .T. ) ;
#49310=ORIENTED_EDGE ( 'NONE', *, *, #58323, .T. ) ;
#49311=EDGE_CURVE ( 'NONE', #77153, #21611, #94663, .T. ) ;
#49312=DIRECTION ( 'NONE',  ( 0.000000000000000000, 0.000000000000000000, -1.000000000000000000 ) ) ;
#49313=DIRECTION ( 'NONE',  ( 0.000000000000000000, -0.000000000000000000, 1.000000000000000000 ) ) ;
#49314=AXIS2_PLACEMENT_3D ( 'NONE', #71958, #33332, #22866 ) ;
#49315=LINE ( 'NONE', #59118, #13724 ) ;
#49316=CARTESIAN_POINT ( 'NONE',  ( -1.250000000000035749, 2.500000000000000000, -7.188010851410854052 ) ) ;
#49317=AXIS2_PLACEMENT_3D ( 'NONE', #90338, #19695, #89715 ) ;
#49318=DIRECTION ( 'NONE',  ( 0.000000000000000000, 0.000000000000000000, -1.000000000000000000 ) ) ;
#49319=FACE_OUTER_BOUND ( 'NONE', #35657, .T. ) ;
#49320=LINE ( 'NONE', #59123, #72880 ) ;
#49321=CARTESIAN_POINT ( 'NONE',  ( 10.84999999999990905, 12.50000000000000000, -6.495190528383302464 ) ) ;
#49322=DIRECTION ( 'NONE',  ( -0.000000000000000000, -1.000000000000000000, -0.000000000000000000 ) ) ;
#49323=CARTESIAN_POINT ( 'NONE',  ( 6.649999999999931966, 12.50000000000000000, -5.867463478539787225 ) ) ;
#49324=AXIS2_PLACEMENT_3D ( 'NONE', #47343, #47990, #97716 ) ;
#49325=ORIENTED_EDGE ( 'NONE', *, *, #100274, .F. ) ;
#49326=VERTEX_POINT ( 'NONE', #124780 ) ;
#49327=CONICAL_SURFACE ( 'NONE', #114142, 0.1000000000000002554, 0.003490658503988666988 ) ;
#49328=VERTEX_POINT ( 'NONE', #25265 ) ;
#49329=VERTEX_POINT ( 'NONE', #35130 ) ;
#49330=CARTESIAN_POINT ( 'NONE',  ( 17.50000000000000355, -2.500000000000059064, -3.093179327514925081 ) ) ;
#49331=DIRECTION ( 'NONE',  ( 0.000000000000000000, -0.000000000000000000, 1.000000000000000000 ) ) ;
#49333=ORIENTED_EDGE ( 'NONE', *, *, #83995, .T. ) ;
#49334=ORIENTED_EDGE ( 'NONE', *, *, #78766, .T. ) ;
#49335=ORIENTED_EDGE ( 'NONE', *, *, #84854, .F. ) ;
#49336=CARTESIAN_POINT ( 'NONE',  ( -3.950000000000025491, 2.500000000000000000, 6.248780366869521430 ) ) ;
#49337=DIRECTION ( 'NONE',  ( 0.000000000000000000, 0.000000000000000000, 1.000000000000000000 ) ) ;
#49338=DIRECTION ( 'NONE',  ( 0.000000000000000000, 0.000000000000000000, 1.000000000000000000 ) ) ;
#49339=CARTESIAN_POINT ( 'NONE',  ( -11.05000000000000249, 12.50000000000000000, -1.883746621131359600 ) ) ;
#49340=CARTESIAN_POINT ( 'NONE',  ( -8.350000000000013856, 12.50000000000000000, -5.802370205355744659 ) ) ;
#49341=DIRECTION ( 'NONE',  ( 0.000000000000000000, -0.9999939076577903929, 0.003490651415223739937 ) ) ;
#49342=DIRECTION ( 'NONE',  ( 0.000000000000000000, 0.000000000000000000, 1.000000000000000000 ) ) ;
#49343=ORIENTED_EDGE ( 'NONE', *, *, #9125, .T. ) ;
#49344=DIRECTION ( 'NONE',  ( 0.000000000000000000, 0.000000000000000000, -1.000000000000000000 ) ) ;
#49345=EDGE_LOOP ( 'NONE', ( #112301, #4628 ) ) ;
#49346=ADVANCED_FACE ( 'NONE', ( #75035 ), #114669, .T. ) ;
#49347=AXIS2_PLACEMENT_3D ( 'NONE', #47362, #87268, #127221 ) ;
#49348=ORIENTED_EDGE ( 'NONE', *, *, #18456, .F. ) ;
#49349=VERTEX_POINT ( 'NONE', #103203 ) ;
#49350=CIRCLE ( 'NONE', #80730, 0.09999999999999982514 ) ;
#49351=EDGE_CURVE ( 'NONE', #11954, #118880, #27214, .T. ) ;
#49352=CARTESIAN_POINT ( 'NONE',  ( -13.09999999999999076, 2.500000000000000000, 4.776537180435972196 ) ) ;
#49353=EDGE_LOOP ( 'NONE', ( #77562, #66023 ) ) ;
#49354=VERTEX_POINT ( 'NONE', #37054 ) ;
#49355=CARTESIAN_POINT ( 'NONE',  ( 6.899999999999928413, 12.50000000000000000, 3.983716857408420964 ) ) ;
#49356=EDGE_CURVE ( 'NONE', #10762, #108113, #47783, .T. ) ;
#49357=CARTESIAN_POINT ( 'NONE',  ( 13.14999999999990088, 2.500000000000000000, 2.511473670974873507 ) ) ;
#49358=CARTESIAN_POINT ( 'NONE',  ( -2.950000000000030376, 12.50000000000000000, 6.495190528383297135 ) ) ;
#49359=CARTESIAN_POINT ( 'NONE',  ( -10.60000000000000142, 12.50000000000000000, 3.983716857408420964 ) ) ;
#49360=CARTESIAN_POINT ( 'NONE',  ( -10.85000000000000142, 2.500000000000000000, -7.188010851410850499 ) ) ;
#49361=EDGE_LOOP ( 'NONE', ( #11164, #81998, #5625, #116468 ) ) ;
#49362=DIRECTION ( 'NONE',  ( 0.000000000000000000, 0.000000000000000000, 1.000000000000000000 ) ) ;
#49364=ORIENTED_EDGE ( 'NONE', *, *, #127886, .T. ) ;
#49365=CARTESIAN_POINT ( 'NONE',  ( -1.450000000000035927, 12.50000000000000000, -1.753560074763288679 ) ) ;
#49366=CIRCLE ( 'NONE', #93262, 0.1000000000000002554 ) ;
#49369=DIRECTION ( 'NONE',  ( 0.000000000000000000, 0.000000000000000000, 1.000000000000000000 ) ) ;
#49370=VECTOR ( 'NONE', #30724, 1000.000000000000000 ) ;
#49371=ORIENTED_EDGE ( 'NONE', *, *, #28587, .T. ) ;
#49372=DIRECTION ( 'NONE',  ( 0.000000000000000000, 0.000000000000000000, 1.000000000000000000 ) ) ;
#49373=DIRECTION ( 'NONE',  ( 0.000000000000000000, 0.000000000000000000, 1.000000000000000000 ) ) ;
#49374=ORIENTED_EDGE ( 'NONE', *, *, #80298, .T. ) ;
#49375=DIRECTION ( 'NONE',  ( 0.000000000000000000, 0.000000000000000000, -1.000000000000000000 ) ) ;
#49376=ORIENTED_EDGE ( 'NONE', *, *, #52657, .T. ) ;
#49377=ORIENTED_EDGE ( 'NONE', *, *, #46421, .F. ) ;
#49378=PLANE ( 'NONE',  #16234 ) ;
#49379=DIRECTION ( 'NONE',  ( 0.000000000000000000, 1.000000000000000000, 0.000000000000000000 ) ) ;
#49381=AXIS2_PLACEMENT_3D ( 'NONE', #124955, #25438, #5802 ) ;
#49382=DIRECTION ( 'NONE',  ( 0.000000000000000000, 0.000000000000000000, 1.000000000000000000 ) ) ;
#49383=LINE ( 'NONE', #81415, #39530 ) ;
#49384=ORIENTED_EDGE ( 'NONE', *, *, #18401, .T. ) ;
#49385=CIRCLE ( 'NONE', #53856, 0.1000000000000002554 ) ;
#49387=AXIS2_PLACEMENT_3D ( 'NONE', #64100, #14964, #83745 ) ;
#49388=AXIS2_PLACEMENT_3D ( 'NONE', #91767, #110753, #32872 ) ;
#49389=ORIENTED_EDGE ( 'NONE', *, *, #90027, .T. ) ;
#49390=DIRECTION ( 'NONE',  ( 0.000000000000000000, 1.000000000000000000, 0.000000000000000000 ) ) ;
#49392=CONICAL_SURFACE ( 'NONE', #3311, 0.1000000000000002554, 0.003490658503988666988 ) ;
#49393=ADVANCED_FACE ( 'NONE', ( #8852 ), #45732, .T. ) ;
#49394=DIRECTION ( 'NONE',  ( -0.000000000000000000, -1.000000000000000000, -0.000000000000000000 ) ) ;
#49395=DIRECTION ( 'NONE',  ( 0.000000000000000000, 0.000000000000000000, 1.000000000000000000 ) ) ;
#49396=CARTESIAN_POINT ( 'NONE',  ( 7.099999999999928590, 2.500000000000000000, 4.330127018922196314 ) ) ;
#49397=EDGE_CURVE ( 'NONE', #71725, #2601, #16458, .T. ) ;
#49398=DIRECTION ( 'NONE',  ( -0.000000000000000000, -1.000000000000000000, -0.000000000000000000 ) ) ;
#49399=DIRECTION ( 'NONE',  ( 0.000000000000000000, -0.000000000000000000, 1.000000000000000000 ) ) ;
#49400=EDGE_LOOP ( 'NONE', ( #108259, #48684 ) ) ;
#49401=AXIS2_PLACEMENT_3D ( 'NONE', #124913, #7047, #7698 ) ;
#49403=AXIS2_PLACEMENT_3D ( 'NONE', #60751, #119027, #20177 ) ;
#49404=AXIS2_PLACEMENT_3D ( 'NONE', #115261, #67452, #106751 ) ;
#49405=DIRECTION ( 'NONE',  ( 0.000000000000000000, 0.000000000000000000, 1.000000000000000000 ) ) ;
#49406=EDGE_CURVE ( 'NONE', #119162, #50950, #5995, .T. ) ;
#49407=ORIENTED_EDGE ( 'NONE', *, *, #68631, .F. ) ;
#49408=DIRECTION ( 'NONE',  ( 0.000000000000000000, 1.000000000000000000, 0.000000000000000000 ) ) ;
#49409=VERTEX_POINT ( 'NONE', #117498 ) ;
#49410=ORIENTED_EDGE ( 'NONE', *, *, #92749, .T. ) ;
#49411=DIRECTION ( 'NONE',  ( -0.000000000000000000, -1.000000000000000000, -0.000000000000000000 ) ) ;
#49412=EDGE_LOOP ( 'NONE', ( #70532, #100273 ) ) ;
#49413=DIRECTION ( 'NONE',  ( 0.000000000000000000, 0.000000000000000000, 1.000000000000000000 ) ) ;
#49414=FACE_OUTER_BOUND ( 'NONE', #121774, .T. ) ;
#49415=ORIENTED_EDGE ( 'NONE', *, *, #107631, .F. ) ;
#49416=CARTESIAN_POINT ( 'NONE',  ( -1.900000000000034106, 2.500000000000000000, 0.2464101615137735679 ) ) ;
#49417=FACE_OUTER_BOUND ( 'NONE', #118905, .T. ) ;
#49418=ORIENTED_EDGE ( 'NONE', *, *, #28434, .F. ) ;
#49419=DIRECTION ( 'NONE',  ( 0.000000000000000000, -0.000000000000000000, 1.000000000000000000 ) ) ;
#49420=DIRECTION ( 'NONE',  ( 0.000000000000000000, 0.000000000000000000, 1.000000000000000000 ) ) ;
#49421=VERTEX_POINT ( 'NONE', #16087 ) ;
#49422=ADVANCED_FACE ( 'NONE', ( #98517 ), #79188, .T. ) ;
#49423=AXIS2_PLACEMENT_3D ( 'NONE', #44635, #115270, #25620 ) ;
#49424=VERTEX_POINT ( 'NONE', #116872 ) ;
#49425=AXIS2_PLACEMENT_3D ( 'NONE', #82394, #61467, #21525 ) ;
#49426=ORIENTED_EDGE ( 'NONE', *, *, #54930, .T. ) ;
#49427=FACE_OUTER_BOUND ( 'NONE', #25255, .T. ) ;
#49428=CARTESIAN_POINT ( 'NONE',  ( -5.000000000000024869, 12.50000000000000000, -5.022947341949754119 ) ) ;
#49429=DIRECTION ( 'NONE',  ( -4.274815082592931898E-19, -0.9999939076577903929, -0.003490651415223739937 ) ) ;
#49430=EDGE_CURVE ( 'NONE', #32296, #63903, #62464, .T. ) ;
#49431=EDGE_CURVE ( 'NONE', #107157, #86066, #93938, .T. ) ;
#49432=FACE_BOUND ( 'NONE', #53225, .T. ) ;
#49433=VERTEX_POINT ( 'NONE', #96584 ) ;
#49434=ADVANCED_FACE ( 'NONE', ( #88719 ), #6269, .T. ) ;
#49435=EDGE_CURVE ( 'NONE', #83925, #44623, #56023, .T. ) ;
#49436=CARTESIAN_POINT ( 'NONE',  ( -5.400000000000019895, 2.500000000000000000, 4.330127018922196314 ) ) ;
#49437=DIRECTION ( 'NONE',  ( -0.000000000000000000, 1.000000000000000000, -0.000000000000000000 ) ) ;
#49438=VERTEX_POINT ( 'NONE', #126718 ) ;
#49439=CONICAL_SURFACE ( 'NONE', #45323, 0.09999999999999982514, 0.003490658503988666988 ) ;
#49440=CONICAL_SURFACE ( 'NONE', #66135, 0.1000000000000002554, 0.003490658503988666988 ) ;
#49441=CARTESIAN_POINT ( 'NONE',  ( -10.65000000000000391, 12.50000000000000000, -6.148780366869522673 ) ) ;
#49442=CARTESIAN_POINT ( 'NONE',  ( 16.56576425165007649, 1.499999999999997113, 6.084390597445792359 ) ) ;
#49443=ADVANCED_FACE ( 'NONE', ( #27868 ), #73006, .T. ) ;
#49444=CARTESIAN_POINT ( 'NONE',  ( 10.64999999999991331, 2.500000000000000000, -1.718653347947325827 ) ) ;
#49445=DIRECTION ( 'NONE',  ( 0.000000000000000000, -0.000000000000000000, 1.000000000000000000 ) ) ;
#49446=CARTESIAN_POINT ( 'NONE',  ( 12.04999999999990834, 2.500000000000000000, -2.265063509461101798 ) ) ;
#49447=EDGE_CURVE ( 'NONE', #13831, #122621, #121030, .T. ) ;
#49448=DIRECTION ( 'NONE',  ( 0.000000000000000000, -0.000000000000000000, 1.000000000000000000 ) ) ;
#49449=PLANE ( 'NONE',  #110971 ) ;
#49450=VECTOR ( 'NONE', #93801, 1000.000000000000000 ) ;
#49451=CIRCLE ( 'NONE', #78695, 0.06509327318403745899 ) ;
#49452=CIRCLE ( 'NONE', #30675, 0.09999999999999982514 ) ;
#49453=EDGE_CURVE ( 'NONE', #41372, #27226, #110656, .T. ) ;
#49454=ORIENTED_EDGE ( 'NONE', *, *, #59969, .F. ) ;
#49455=VERTEX_POINT ( 'NONE', #108352 ) ;
#49456=ORIENTED_EDGE ( 'NONE', *, *, #102783, .T. ) ;
#49457=VERTEX_POINT ( 'NONE', #38346 ) ;
#49458=VERTEX_POINT ( 'NONE', #78277 ) ;
#49459=CARTESIAN_POINT ( 'NONE',  ( -1.700000000000034817, 12.50000000000000000, -0.06509327318403980434 ) ) ;
#49460=DIRECTION ( 'NONE',  ( 0.000000000000000000, 0.000000000000000000, 1.000000000000000000 ) ) ;
#49461=ORIENTED_EDGE ( 'NONE', *, *, #105912, .T. ) ;
#49462=EDGE_CURVE ( 'NONE', #20554, #41081, #12357, .T. ) ;
#49463=FACE_BOUND ( 'NONE', #29452, .T. ) ;
#49464=EDGE_CURVE ( 'NONE', #32613, #52515, #70946, .T. ) ;
#49465=CARTESIAN_POINT ( 'NONE',  ( 6.649999999999928413, 2.500000000000000000, 1.572243186433545548 ) ) ;
#49466=DIRECTION ( 'NONE',  ( -0.000000000000000000, -1.000000000000000000, -0.000000000000000000 ) ) ;
#49467=CARTESIAN_POINT ( 'NONE',  ( 3.099999999999945466, 12.50000000000000000, -3.983716857408426293 ) ) ;
#49468=FACE_OUTER_BOUND ( 'NONE', #3592, .T. ) ;
#49469=DIRECTION ( 'NONE',  ( 0.000000000000000000, 1.000000000000000000, 0.000000000000000000 ) ) ;
#49470=CARTESIAN_POINT ( 'NONE',  ( 1.049999999999954525, 12.50000000000000000, 1.818653347947321475 ) ) ;
#49471=CIRCLE ( 'NONE', #89154, 0.1000000000000000472 ) ;
#49472=EDGE_LOOP ( 'NONE', ( #102431, #94586, #119839, #33036 ) ) ;
#49473=ORIENTED_EDGE ( 'NONE', *, *, #31854, .T. ) ;
#49474=AXIS2_PLACEMENT_3D ( 'NONE', #69028, #70332, #38974 ) ;
#49475=ORIENTED_EDGE ( 'NONE', *, *, #63034, .T. ) ;
#49476=EDGE_LOOP ( 'NONE', ( #63425, #89381 ) ) ;
#49477=CARTESIAN_POINT ( 'NONE',  ( 11.75764115802644660, 2.500000000000000000, 7.679135278744413817 ) ) ;
#49478=CONICAL_SURFACE ( 'NONE', #122623, 0.09999999999999999167, 0.003490658503988666988 ) ;
#49479=CARTESIAN_POINT ( 'NONE',  ( 17.50000000000000000, -2.500000000000000000, -3.999999999999998224 ) ) ;
#49480=EDGE_LOOP ( 'NONE', ( #75606, #35477, #62674, #86650 ) ) ;
#49481=CARTESIAN_POINT ( 'NONE',  ( 7.299999999999927880, 2.500000000000000000, 3.883716857408421319 ) ) ;
#49482=AXIS2_PLACEMENT_3D ( 'NONE', #75339, #55067, #88200 ) ;
#49483=AXIS2_PLACEMENT_3D ( 'NONE', #94334, #45256, #64240 ) ;
#49484=CARTESIAN_POINT ( 'NONE',  ( -9.800000000000006040, 2.500000000000000000, 4.576537180435972019 ) ) ;
#49485=CIRCLE ( 'NONE', #122628, 0.1000000000000000472 ) ;
#49486=DIRECTION ( 'NONE',  ( 0.000000000000000000, 0.000000000000000000, 1.000000000000000000 ) ) ;
#49488=CARTESIAN_POINT ( 'NONE',  ( 6.449999999999933564, 2.500000000000000000, -6.741600689897078169 ) ) ;
#49489=FACE_OUTER_BOUND ( 'NONE', #25623, .T. ) ;
#49490=PLANE ( 'NONE',  #68442 ) ;
#49491=ORIENTED_EDGE ( 'NONE', *, *, #63612, .F. ) ;
#49492=DIRECTION ( 'NONE',  ( -0.000000000000000000, 1.000000000000000000, -0.000000000000000000 ) ) ;
#49493=AXIS2_PLACEMENT_3D ( 'NONE', #88850, #31235, #85300 ) ;
#49494=EDGE_LOOP ( 'NONE', ( #45953, #77295 ) ) ;
#49495=EDGE_CURVE ( 'NONE', #18199, #1500, #16542, .T. ) ;
#49496=CIRCLE ( 'NONE', #91329, 0.09999999999999982514 ) ;
#49497=AXIS2_PLACEMENT_3D ( 'NONE', #109991, #58326, #129012 ) ;
#49498=VERTEX_POINT ( 'NONE', #86775 ) ;
#49499=PLANE ( 'NONE',  #71965 ) ;
#49500=EDGE_CURVE ( 'NONE', #101537, #53806, #52086, .T. ) ;
#49501=CARTESIAN_POINT ( 'NONE',  ( -7.700000000000014388, 2.500000000000000000, -4.676537180435977881 ) ) ;
#49502=DIRECTION ( 'NONE',  ( 0.000000000000000000, 1.000000000000000000, 0.000000000000000000 ) ) ;
#49503=EDGE_LOOP ( 'NONE', ( #115595, #104295 ) ) ;
#49504=ORIENTED_EDGE ( 'NONE', *, *, #64210, .T. ) ;
#49505=LINE ( 'NONE', #29846, #5805 ) ;
#49506=DIRECTION ( 'NONE',  ( -4.274815082592931898E-19, -0.9999939076577903929, -0.003490651415223739937 ) ) ;
#49507=CARTESIAN_POINT ( 'NONE',  ( 2.099999999999948574, 12.50000000000000000, 3.572213422710607489 ) ) ;
#49508=ORIENTED_EDGE ( 'NONE', *, *, #89171, .T. ) ;
#49509=CARTESIAN_POINT ( 'NONE',  ( 6.449999999999928235, 12.50000000000000000, 2.446380397790835826 ) ) ;
#49510=EDGE_LOOP ( 'NONE', ( #110638, #106823, #37989, #97161 ) ) ;
#49511=CARTESIAN_POINT ( 'NONE',  ( 2.099999999999950351, 12.50000000000000000, -0.6928203230275541413 ) ) ;
#49512=ORIENTED_EDGE ( 'NONE', *, *, #37021, .T. ) ;
#49513=CARTESIAN_POINT ( 'NONE',  ( -1.700000000000034817, 2.500000000000000000, -2.385244779468109755E-15 ) ) ;
#49514=LINE ( 'NONE', #40990, #102756 ) ;
#49515=DIRECTION ( 'NONE',  ( 0.000000000000000000, -0.000000000000000000, 1.000000000000000000 ) ) ;
#49516=CARTESIAN_POINT ( 'NONE',  ( -4.150000000000027889, 12.50000000000000000, -7.188010851410854052 ) ) ;
#49517=ORIENTED_EDGE ( 'NONE', *, *, #35268, .F. ) ;
#49518=FACE_OUTER_BOUND ( 'NONE', #86267, .T. ) ;
#49519=AXIS2_PLACEMENT_3D ( 'NONE', #86723, #74489, #124239 ) ;
#49520=ORIENTED_EDGE ( 'NONE', *, *, #28007, .F. ) ;
#49521=EDGE_LOOP ( 'NONE', ( #103823, #34540 ) ) ;
#49522=CARTESIAN_POINT ( 'NONE',  ( -0.4500000000000397571, 12.50000000000000000, -2.165063509461101710 ) ) ;
#49523=CARTESIAN_POINT ( 'NONE',  ( 15.19999999999989093, 2.500000000000000000, 0.3464101615137735735 ) ) ;
#49524=CARTESIAN_POINT ( 'NONE',  ( 18.09027855933934603, 2.526462839860887488, 2.685672775344559504 ) ) ;
#49525=LINE ( 'NONE', #31182, #31258 ) ;
#49526=DIRECTION ( 'NONE',  ( 0.000000000000000000, 0.000000000000000000, 1.000000000000000000 ) ) ;
#49527=VECTOR ( 'NONE', #7189, 1000.000000000000000 ) ;
#49528=DIRECTION ( 'NONE',  ( -0.000000000000000000, -1.000000000000000000, -0.000000000000000000 ) ) ;
#49529=VECTOR ( 'NONE', #82607, 1000.000000000000000 ) ;
#49530=EDGE_CURVE ( 'NONE', #22326, #22783, #24886, .T. ) ;
#49531=CARTESIAN_POINT ( 'NONE',  ( -5.400000000000019895, 2.500000000000000000, 3.637306695894644726 ) ) ;
#49532=DIRECTION ( 'NONE',  ( -4.274815082592931898E-19, -0.9999939076577903929, -0.003490651415223739937 ) ) ;
#49533=DIRECTION ( 'NONE',  ( 0.000000000000000000, 1.000000000000000000, 0.000000000000000000 ) ) ;
#49534=CIRCLE ( 'NONE', #128964, 0.06509327318403745899 ) ;
#49535=CIRCLE ( 'NONE', #18116, 0.06509327318403745899 ) ;
#49536=CONICAL_SURFACE ( 'NONE', #51593, 0.1000000000000002554, 0.003490658503988666988 ) ;
#49537=EDGE_CURVE ( 'NONE', #29893, #29014, #69727, .T. ) ;
#49538=CIRCLE ( 'NONE', #101757, 0.1000000000000000472 ) ;
#49539=ORIENTED_EDGE ( 'NONE', *, *, #36254, .F. ) ;
#49541=EDGE_CURVE ( 'NONE', #80196, #92392, #313, .T. ) ;
#49542=CARTESIAN_POINT ( 'NONE',  ( -11.64999999999999680, 2.500000000000000000, 2.265063509461097357 ) ) ;
#49543=FACE_OUTER_BOUND ( 'NONE', #129427, .T. ) ;
#49544=ADVANCED_FACE ( 'NONE', ( #128681 ), #47888, .T. ) ;
#49545=PLANE ( 'NONE',  #71519 ) ;
#49546=DIRECTION ( 'NONE',  ( -0.000000000000000000, -1.000000000000000000, -0.000000000000000000 ) ) ;
#49547=ORIENTED_EDGE ( 'NONE', *, *, #74992, .T. ) ;
#49548=CARTESIAN_POINT ( 'NONE',  ( -0.2000000000000399791, 2.500000000000000000, -4.676537180435977881 ) ) ;
#49549=CARTESIAN_POINT ( 'NONE',  ( 12.29999999999990656, 12.50000000000000000, -4.676537180435977881 ) ) ;
#49550=LINE ( 'NONE', #118919, #4523 ) ;
#49551=ORIENTED_EDGE ( 'NONE', *, *, #60657, .T. ) ;
#49552=EDGE_CURVE ( 'NONE', #24359, #115574, #127299, .T. ) ;
#49553=CIRCLE ( 'NONE', #41159, 0.06509327318403745899 ) ;
#49554=CIRCLE ( 'NONE', #41242, 0.06509327318403743123 ) ;
#49555=EDGE_LOOP ( 'NONE', ( #124644, #62224, #49212, #104317 ) ) ;
#49556=CONICAL_SURFACE ( 'NONE', #30782, 0.1000000000000002554, 0.003490658503988666988 ) ;
#49557=CARTESIAN_POINT ( 'NONE',  ( 1.049999999999954969, 2.500000000000000000, -6.741600689897077281 ) ) ;
#49558=CIRCLE ( 'NONE', #72549, 0.1000000000000002554 ) ;
#49559=EDGE_LOOP ( 'NONE', ( #110531, #67326, #81021, #66876 ) ) ;
#49561=ORIENTED_EDGE ( 'NONE', *, *, #74581, .F. ) ;
#49562=DIRECTION ( 'NONE',  ( -4.274815082592931898E-19, -0.9999939076577903929, -0.003490651415223739937 ) ) ;
#49563=CARTESIAN_POINT ( 'NONE',  ( 14.34999999999989662, 2.500000000000000000, 2.511473670974873507 ) ) ;
#49564=FACE_OUTER_BOUND ( 'NONE', #35427, .T. ) ;
#49565=AXIS2_PLACEMENT_3D ( 'NONE', #52180, #92090, #12870 ) ;
#49566=DIRECTION ( 'NONE',  ( -4.274815082592931898E-19, -0.9999939076577903929, -0.003490651415223739937 ) ) ;
#49567=ORIENTED_EDGE ( 'NONE', *, *, #9383, .F. ) ;
#49568=VECTOR ( 'NONE', #61631, 1000.000000000000000 ) ;
#49570=EDGE_LOOP ( 'NONE', ( #23610, #90687, #31176, #89184 ) ) ;
#49571=CARTESIAN_POINT ( 'NONE',  ( -0.6500000000000398792, 12.50000000000000000, -6.841600689897078702 ) ) ;
#49572=CARTESIAN_POINT ( 'NONE',  ( 15.24415751722802526, 2.474878586408650438, 4.460068884075454321 ) ) ;
#49573=CARTESIAN_POINT ( 'NONE',  ( 7.299999999999926104, 12.50000000000000000, -0.2813168883297408329 ) ) ;
#49574=CONICAL_SURFACE ( 'NONE', #80872, 0.1000000000000002554, 0.003490658503988666988 ) ;
#49575=CARTESIAN_POINT ( 'NONE',  ( 1.049999999999954525, 12.50000000000000000, 1.818653347947321475 ) ) ;
#49576=CIRCLE ( 'NONE', #45374, 0.06509327318403745899 ) ;
#49577=ORIENTED_EDGE ( 'NONE', *, *, #95664, .T. ) ;
#49578=EDGE_CURVE ( 'NONE', #100057, #79205, #102255, .T. ) ;
#49579=AXIS2_PLACEMENT_3D ( 'NONE', #10813, #110960, #43549 ) ;
#49580=AXIS2_PLACEMENT_3D ( 'NONE', #45767, #65385, #126900 ) ;
#49581=ORIENTED_EDGE ( 'NONE', *, *, #123623, .T. ) ;
#49582=ORIENTED_EDGE ( 'NONE', *, *, #5483, .F. ) ;
#49583=VERTEX_POINT ( 'NONE', #61197 ) ;
#49584=VERTEX_POINT ( 'NONE', #39651 ) ;
#49585=CARTESIAN_POINT ( 'NONE',  ( -10.20000000000000462, 2.500000000000000000, -4.676537180435973440 ) ) ;
#49586=DIRECTION ( 'NONE',  ( -0.000000000000000000, 1.000000000000000000, -0.000000000000000000 ) ) ;
#49587=FACE_OUTER_BOUND ( 'NONE', #64968, .T. ) ;
#49588=EDGE_CURVE ( 'NONE', #42202, #10139, #20635, .T. ) ;
#49589=FACE_BOUND ( 'NONE', #35880, .T. ) ;
#49590=DIRECTION ( 'NONE',  ( -0.000000000000000000, -1.000000000000000000, -0.000000000000000000 ) ) ;
#49592=EDGE_CURVE ( 'NONE', #120278, #125645, #29174, .T. ) ;
#49594=DIRECTION ( 'NONE',  ( 0.000000000000000000, 0.000000000000000000, 1.000000000000000000 ) ) ;
#49595=ADVANCED_FACE ( 'NONE', ( #19988 ), #41640, .T. ) ;
#49596=DIRECTION ( 'NONE',  ( 0.000000000000000000, 0.000000000000000000, 1.000000000000000000 ) ) ;
#49597=EDGE_CURVE ( 'NONE', #58191, #97339, #110920, .T. ) ;
#49598=DIRECTION ( 'NONE',  ( -0.000000000000000000, 1.000000000000000000, -0.000000000000000000 ) ) ;
#49599=EDGE_CURVE ( 'NONE', #74569, #66767, #91782, .T. ) ;
#49600=AXIS2_PLACEMENT_3D ( 'NONE', #22118, #52199, #79095 ) ;
#49601=LINE ( 'NONE', #8353, #24060 ) ;
#49602=ADVANCED_FACE ( 'NONE', ( #108982 ), #1892, .T. ) ;
#49603=DIRECTION ( 'NONE',  ( -0.000000000000000000, 1.000000000000000000, -0.000000000000000000 ) ) ;
#49604=EDGE_CURVE ( 'NONE', #119959, #88710, #125236, .T. ) ;
#49605=EDGE_LOOP ( 'NONE', ( #51281, #25938 ) ) ;
#49606=ORIENTED_EDGE ( 'NONE', *, *, #87238, .T. ) ;
#49607=VERTEX_POINT ( 'NONE', #49465 ) ;
#49608=ORIENTED_EDGE ( 'NONE', *, *, #8614, .F. ) ;
#49609=CARTESIAN_POINT ( 'NONE',  ( 2.099999999999950351, 2.500000000000000000, -4.430127018922202176 ) ) ;
#49610=PLANE ( 'NONE',  #109293 ) ;
#49611=FACE_BOUND ( 'NONE', #47177, .T. ) ;
#49612=EDGE_CURVE ( 'NONE', #116018, #118459, #4032, .T. ) ;
#49613=DIRECTION ( 'NONE',  ( -0.000000000000000000, -1.000000000000000000, -0.000000000000000000 ) ) ;
#49614=AXIS2_PLACEMENT_3D ( 'NONE', #1808, #50934, #10968 ) ;
#49615=VECTOR ( 'NONE', #60507, 1000.000000000000000 ) ;
#49616=ORIENTED_EDGE ( 'NONE', *, *, #63284, .F. ) ;
#49618=DIRECTION ( 'NONE',  ( -4.274815082592931898E-19, -0.9999939076577903929, -0.003490651415223739937 ) ) ;
#49619=CARTESIAN_POINT ( 'NONE',  ( 13.34999999999989662, 2.500000000000000000, -2.065063509461102065 ) ) ;
#49620=FACE_OUTER_BOUND ( 'NONE', #43629, .T. ) ;
#49621=ORIENTED_EDGE ( 'NONE', *, *, #98739, .F. ) ;
#49622=DIRECTION ( 'NONE',  ( 0.000000000000000000, 0.000000000000000000, -1.000000000000000000 ) ) ;
#49623=CIRCLE ( 'NONE', #53803, 0.1000000000000002554 ) ;
#49624=VECTOR ( 'NONE', #12598, 1000.000000000000000 ) ;
#49625=ORIENTED_EDGE ( 'NONE', *, *, #13084, .F. ) ;
#49626=EDGE_LOOP ( 'NONE', ( #37446, #85560 ) ) ;
#49627=CARTESIAN_POINT ( 'NONE',  ( 10.79999999999991012, 2.500000000000000000, 4.430127018922196847 ) ) ;
#49628=DIRECTION ( 'NONE',  ( -0.000000000000000000, 1.000000000000000000, -0.000000000000000000 ) ) ;
#49629=EDGE_LOOP ( 'NONE', ( #125150, #33913, #88769, #37746 ) ) ;
#49631=CONICAL_SURFACE ( 'NONE', #95585, 0.1000000000000002554, 0.003490658503988666988 ) ;
#49632=CIRCLE ( 'NONE', #85208, 0.09999999999999982514 ) ;
#49633=CARTESIAN_POINT ( 'NONE',  ( -6.250000000000019540, 2.500000000000000000, -7.288010851410854585 ) ) ;
#49634=DIRECTION ( 'NONE',  ( -4.274815082592931898E-19, -0.9999939076577903929, -0.003490651415223739937 ) ) ;
#49635=ORIENTED_EDGE ( 'NONE', *, *, #75707, .F. ) ;
#49636=DIRECTION ( 'NONE',  ( 0.000000000000000000, 0.000000000000000000, 1.000000000000000000 ) ) ;
#49637=VERTEX_POINT ( 'NONE', #29803 ) ;
#49638=CARTESIAN_POINT ( 'NONE',  ( -6.850000000000013856, 2.500000000000000000, 2.611473670974873151 ) ) ;
#49639=VERTEX_POINT ( 'NONE', #99844 ) ;
#49641=FACE_BOUND ( 'NONE', #19905, .T. ) ;
#49642=CIRCLE ( 'NONE', #83368, 0.1000000000000002554 ) ;
#49643=ORIENTED_EDGE ( 'NONE', *, *, #47499, .F. ) ;
#49644=EDGE_CURVE ( 'NONE', #125681, #33832, #18619, .T. ) ;
#49646=ORIENTED_EDGE ( 'NONE', *, *, #40239, .F. ) ;
#49647=DIRECTION ( 'NONE',  ( 0.000000000000000000, 0.000000000000000000, 1.000000000000000000 ) ) ;
#49648=DIRECTION ( 'NONE',  ( -4.274815082592931898E-19, -0.9999939076577903929, -0.003490651415223739937 ) ) ;
#49649=DIRECTION ( 'NONE',  ( -0.000000000000000000, 1.000000000000000000, -0.000000000000000000 ) ) ;
#49650=DIRECTION ( 'NONE',  ( 0.000000000000000000, 1.000000000000000000, 0.000000000000000000 ) ) ;
#49651=PLANE ( 'NONE',  #66307 ) ;
#49652=AXIS2_PLACEMENT_3D ( 'NONE', #47059, #37244, #54289 ) ;
#49653=ORIENTED_EDGE ( 'NONE', *, *, #51023, .F. ) ;
#49654=ORIENTED_EDGE ( 'NONE', *, *, #43202, .F. ) ;
#49655=ADVANCED_FACE ( 'NONE', ( #31109 ), #10162, .T. ) ;
#49656=ORIENTED_EDGE ( 'NONE', *, *, #41052, .T. ) ;
#49657=CARTESIAN_POINT ( 'NONE',  ( 4.149999999999939959, 2.500000000000000000, -6.495190528383302464 ) ) ;
#49658=AXIS2_PLACEMENT_3D ( 'NONE', #80138, #120060, #62441 ) ;
#49659=CARTESIAN_POINT ( 'NONE',  ( -2.700000000000030820, 2.500000000000000000, 0.4464101615137735513 ) ) ;
#49660=DIRECTION ( 'NONE',  ( 0.000000000000000000, 0.000000000000000000, 1.000000000000000000 ) ) ;
#49661=VERTEX_POINT ( 'NONE', #81484 ) ;
#49662=EDGE_LOOP ( 'NONE', ( #99726, #111475, #1182, #121593 ) ) ;
#49663=ORIENTED_EDGE ( 'NONE', *, *, #52950, .F. ) ;
#49664=CARTESIAN_POINT ( 'NONE',  ( -11.05000000000000071, 2.500000000000000000, -6.941600689897075682 ) ) ;
#49665=CONICAL_SURFACE ( 'NONE', #53749, 0.1000000000000002554, 0.003490658503988666988 ) ;
#49666=CIRCLE ( 'NONE', #53751, 0.1000000000000002554 ) ;
#49667=DIRECTION ( 'NONE',  ( 0.000000000000000000, 0.000000000000000000, 1.000000000000000000 ) ) ;
#49669=CONICAL_SURFACE ( 'NONE', #57968, 0.09999999999999999167, 0.003490658503988666988 ) ;
#49671=DIRECTION ( 'NONE',  ( 0.000000000000000000, -0.9999939076577903929, 0.003490651415223739937 ) ) ;
#49672=DIRECTION ( 'NONE',  ( 0.000000000000000000, 1.000000000000000000, 0.000000000000000000 ) ) ;
#49673=CARTESIAN_POINT ( 'NONE',  ( -0.2000000000000347888, 2.500000000000000000, 0.3464101615137758494 ) ) ;
#49674=CARTESIAN_POINT ( 'NONE',  ( 13.94999999999989448, 2.500000000000000000, -2.611473670974877592 ) ) ;
#49676=AXIS2_PLACEMENT_3D ( 'NONE', #100032, #58187, #98719 ) ;
#49677=CARTESIAN_POINT ( 'NONE',  ( -4.800000000000026468, 2.500000000000000000, -4.576537180435978236 ) ) ;
#49678=ORIENTED_EDGE ( 'NONE', *, *, #58002, .T. ) ;
#49679=ORIENTED_EDGE ( 'NONE', *, *, #81655, .F. ) ;
#49680=CARTESIAN_POINT ( 'NONE',  ( -1.850000000000033396, 12.50000000000000000, -6.841600689897077814 ) ) ;
#49681=VECTOR ( 'NONE', #35648, 1000.000000000000000 ) ;
#49682=CIRCLE ( 'NONE', #1529, 0.06509327318403745899 ) ;
#49683=CARTESIAN_POINT ( 'NONE',  ( 10.39999999999991509, 2.500000000000000000, 0.5928203230275495006 ) ) ;
#49684=EDGE_LOOP ( 'NONE', ( #101744, #28834 ) ) ;
#49685=ORIENTED_EDGE ( 'NONE', *, *, #127482, .T. ) ;
#49686=CARTESIAN_POINT ( 'NONE',  ( 14.14999999999989733, 12.50000000000000000, 2.792790559304612064 ) ) ;
#49687=DIRECTION ( 'NONE',  ( -0.000000000000000000, -1.000000000000000000, -0.000000000000000000 ) ) ;
#49688=CARTESIAN_POINT ( 'NONE',  ( -2.100000000000034284, 2.500000000000000000, 0.09999999999999761857 ) ) ;
#49689=DIRECTION ( 'NONE',  ( -0.000000000000000000, 1.000000000000000000, -0.000000000000000000 ) ) ;
#49690=EDGE_CURVE ( 'NONE', #41939, #55594, #85522, .T. ) ;
#49691=LINE ( 'NONE', #39872, #53257 ) ;
#49692=CARTESIAN_POINT ( 'NONE',  ( -9.550000000000006040, 12.50000000000000000, 2.165063509461097713 ) ) ;
#49693=DIRECTION ( 'NONE',  ( 0.000000000000000000, 0.000000000000000000, -1.000000000000000000 ) ) ;
#49695=LINE ( 'NONE', #59528, #43719 ) ;
#49696=EDGE_CURVE ( 'NONE', #81742, #88394, #82786, .T. ) ;
#49697=ORIENTED_EDGE ( 'NONE', *, *, #116381, .F. ) ;
#49699=ADVANCED_FACE ( 'NONE', ( #3561 ), #114165, .T. ) ;
#49700=ORIENTED_EDGE ( 'NONE', *, *, #73844, .F. ) ;
#49701=ORIENTED_EDGE ( 'NONE', *, *, #93672, .F. ) ;
#49702=ADVANCED_FACE ( 'NONE', ( #13375 ), #89730, .T. ) ;
#49703=DIRECTION ( 'NONE',  ( 0.000000000000000000, -0.000000000000000000, 1.000000000000000000 ) ) ;
#49704=DIRECTION ( 'NONE',  ( 0.000000000000000000, 0.000000000000000000, -1.000000000000000000 ) ) ;
#49705=ORIENTED_EDGE ( 'NONE', *, *, #71297, .F. ) ;
#49706=VECTOR ( 'NONE', #8725, 1000.000000000000000 ) ;
#49707=DIRECTION ( 'NONE',  ( 0.000000000000000000, 0.000000000000000000, 1.000000000000000000 ) ) ;
#49708=AXIS2_PLACEMENT_3D ( 'NONE', #31053, #61133, #91882 ) ;
#49710=ADVANCED_FACE ( 'NONE', ( #112233 ), #56271, .T. ) ;
#49712=CARTESIAN_POINT ( 'NONE',  ( -11.05000000000000071, 2.500000000000000000, 2.411473670974873862 ) ) ;
#49713=EDGE_LOOP ( 'NONE', ( #111226, #120189 ) ) ;
#49714=ADVANCED_FACE ( 'NONE', ( #42875 ), #43781, .T. ) ;
#49715=CARTESIAN_POINT ( 'NONE',  ( 0.6499999999999561684, 2.500000000000000000, -1.718653347947325827 ) ) ;
#49716=AXIS2_PLACEMENT_3D ( 'NONE', #12460, #129216, #62862 ) ;
#49717=DIRECTION ( 'NONE',  ( 0.000000000000000000, 1.000000000000000000, 0.000000000000000000 ) ) ;
#49718=VERTEX_POINT ( 'NONE', #32411 ) ;
#49719=CONICAL_SURFACE ( 'NONE', #95672, 0.1000000000000002554, 0.003490658503988666988 ) ;
#49720=AXIS2_PLACEMENT_3D ( 'NONE', #58502, #8705, #100978 ) ;
#49721=ORIENTED_EDGE ( 'NONE', *, *, #74503, .T. ) ;
#49722=ORIENTED_EDGE ( 'NONE', *, *, #125528, .F. ) ;
#49723=VERTEX_POINT ( 'NONE', #33671 ) ;
#49724=CARTESIAN_POINT ( 'NONE',  ( -13.94999999999998685, 12.50000000000000000, -2.511473670974875727 ) ) ;
#49725=DIRECTION ( 'NONE',  ( 0.000000000000000000, 0.000000000000000000, 1.000000000000000000 ) ) ;
#49726=FACE_OUTER_BOUND ( 'NONE', #62051, .T. ) ;
#49727=AXIS2_PLACEMENT_3D ( 'NONE', #99527, #39331, #49785 ) ;
#49728=ORIENTED_EDGE ( 'NONE', *, *, #47388, .F. ) ;
#49729=AXIS2_PLACEMENT_3D ( 'NONE', #118736, #79477, #10078 ) ;
#49731=DIRECTION ( 'NONE',  ( -0.000000000000000000, 1.000000000000000000, -0.000000000000000000 ) ) ;
#49732=CARTESIAN_POINT ( 'NONE',  ( 5.399999999999933742, 2.500000000000000000, 0.09999999999999761857 ) ) ;
#49733=CARTESIAN_POINT ( 'NONE',  ( -14.99999999999994671, 2.500000000000000000, 0.000000000000000000 ) ) ;
#49734=EDGE_LOOP ( 'NONE', ( #103242, #73821, #113415, #51794 ) ) ;
#49735=CIRCLE ( 'NONE', #1677, 0.06509327318403745899 ) ;
#49736=DIRECTION ( 'NONE',  ( -0.000000000000000000, 1.000000000000000000, -0.000000000000000000 ) ) ;
#49737=AXIS2_PLACEMENT_3D ( 'NONE', #66368, #106296, #56541 ) ;
#49738=ORIENTED_EDGE ( 'NONE', *, *, #11726, .F. ) ;
#49739=EDGE_LOOP ( 'NONE', ( #8918, #114856 ) ) ;
#49740=DIRECTION ( 'NONE',  ( 0.000000000000000000, 1.000000000000000000, 0.000000000000000000 ) ) ;
#49741=DIRECTION ( 'NONE',  ( -4.274815082592931898E-19, -0.9999939076577903929, -0.003490651415223739937 ) ) ;
#49742=FACE_BOUND ( 'NONE', #73172, .T. ) ;
#49743=VECTOR ( 'NONE', #20510, 1000.000000000000000 ) ;
#49744=DIRECTION ( 'NONE',  ( 0.000000000000000000, -0.9999939076577903929, 0.003490651415223739937 ) ) ;
#49745=CARTESIAN_POINT ( 'NONE',  ( 8.099999999999923261, 2.500000000000000000, -3.883716857408426648 ) ) ;
#49746=AXIS2_PLACEMENT_3D ( 'NONE', #62216, #11152, #51108 ) ;
#49747=FACE_OUTER_BOUND ( 'NONE', #7886, .T. ) ;
#49748=CIRCLE ( 'NONE', #35172, 0.06509327318403745899 ) ;
#49749=EDGE_CURVE ( 'NONE', #79243, #22283, #54576, .T. ) ;
#49750=EDGE_LOOP ( 'NONE', ( #99341, #126650, #48734, #60320 ) ) ;
#49751=EDGE_CURVE ( 'NONE', #80732, #114635, #12447, .T. ) ;
#49752=PLANE ( 'NONE',  #67241 ) ;
#49753=CARTESIAN_POINT ( 'NONE',  ( -11.89999999999999503, 2.500000000000000000, 3.983716857408420076 ) ) ;
#49754=CARTESIAN_POINT ( 'NONE',  ( -8.950000000000009948, 2.500000000000000000, -1.918653347947326004 ) ) ;
#49755=ADVANCED_FACE ( 'NONE', ( #15289 ), #25128, .T. ) ;
#49756=AXIS2_PLACEMENT_3D ( 'NONE', #59291, #50738, #69077 ) ;
#49757=LINE ( 'NONE', #90950, #23963 ) ;
#49759=EDGE_CURVE ( 'NONE', #129270, #110798, #93878, .T. ) ;
#49761=AXIS2_PLACEMENT_3D ( 'NONE', #111864, #109267, #81737 ) ;
#49762=DIRECTION ( 'NONE',  ( -0.000000000000000000, 1.000000000000000000, -0.000000000000000000 ) ) ;
#49763=EDGE_CURVE ( 'NONE', #105720, #129537, #37606, .T. ) ;
#49764=VERTEX_POINT ( 'NONE', #23858 ) ;
#49765=EDGE_LOOP ( 'NONE', ( #79838, #42319, #16021, #91199 ) ) ;
#49766=DIRECTION ( 'NONE',  ( 0.000000000000000000, 0.000000000000000000, 1.000000000000000000 ) ) ;
#49767=CIRCLE ( 'NONE', #108233, 0.06509327318403745899 ) ;
#49768=FACE_BOUND ( 'NONE', #17895, .T. ) ;
#49769=DIRECTION ( 'NONE',  ( 0.000000000000000000, -0.9999939076577903929, 0.003490651415223739937 ) ) ;
#49770=EDGE_CURVE ( 'NONE', #94750, #129385, #14583, .T. ) ;
#49772=CIRCLE ( 'NONE', #39319, 0.06509327318403745899 ) ;
#49773=EDGE_CURVE ( 'NONE', #47419, #72591, #85610, .T. ) ;
#49774=DIRECTION ( 'NONE',  ( -0.000000000000000000, -1.000000000000000000, -0.000000000000000000 ) ) ;
#49775=ORIENTED_EDGE ( 'NONE', *, *, #46411, .T. ) ;
#49776=CARTESIAN_POINT ( 'NONE',  ( -10.60000000000000142, 12.50000000000000000, 4.676537180435972552 ) ) ;
#49778=VERTEX_POINT ( 'NONE', #112877 ) ;
#49779=DIRECTION ( 'NONE',  ( -0.000000000000000000, -1.000000000000000000, -0.000000000000000000 ) ) ;
#49780=CARTESIAN_POINT ( 'NONE',  ( -2.300000000000032685, 12.50000000000000000, -4.611443907251940644 ) ) ;
#49781=CARTESIAN_POINT ( 'NONE',  ( 6.449999999999930012, 12.50000000000000000, -1.818653347947326138 ) ) ;
#49782=FACE_OUTER_BOUND ( 'NONE', #110340, .T. ) ;
#49783=ORIENTED_EDGE ( 'NONE', *, *, #96856, .F. ) ;
#49784=PLANE ( 'NONE',  #101048 ) ;
#49785=DIRECTION ( 'NONE',  ( 0.000000000000000000, 0.000000000000000000, -1.000000000000000000 ) ) ;
#49786=VECTOR ( 'NONE', #105329, 1000.000000000000000 ) ;
#49787=CARTESIAN_POINT ( 'NONE',  ( 6.249999999999930722, 12.50000000000000000, 1.407149913249508000 ) ) ;
#49788=CARTESIAN_POINT ( 'NONE',  ( 0.1999999999999562961, 2.500000000000000000, 4.676537180435972552 ) ) ;
#49789=EDGE_LOOP ( 'NONE', ( #43751, #122665, #81726, #54689 ) ) ;
#49790=AXIS2_PLACEMENT_3D ( 'NONE', #102563, #13539, #60726 ) ;
#49791=EDGE_LOOP ( 'NONE', ( #2410, #56800, #3973, #39134 ) ) ;
#49792=DIRECTION ( 'NONE',  ( -0.000000000000000000, 1.000000000000000000, -0.000000000000000000 ) ) ;
#49793=EDGE_LOOP ( 'NONE', ( #35878, #21003 ) ) ;
#49794=CARTESIAN_POINT ( 'NONE',  ( -3.100000000000028511, 2.500000000000000000, -4.676537180435977881 ) ) ;
#49795=CARTESIAN_POINT ( 'NONE',  ( 87.50000000000000000, -7.499999999999999112, -0.6928095518838432998 ) ) ;
#49796=VECTOR ( 'NONE', #98903, 1000.000000000000000 ) ;
#49797=AXIS2_PLACEMENT_3D ( 'NONE', #128453, #129103, #58417 ) ;
#49798=CARTESIAN_POINT ( 'NONE',  ( -13.14999999999999147, 12.50000000000000000, -1.753560074763286458 ) ) ;
#49799=ORIENTED_EDGE ( 'NONE', *, *, #119973, .T. ) ;
#49800=DIRECTION ( 'NONE',  ( 0.000000000000000000, 0.000000000000000000, -1.000000000000000000 ) ) ;
#49801=CARTESIAN_POINT ( 'NONE',  ( 0.8499999999999545697, 2.500000000000000000, -1.372243186433550033 ) ) ;
#49802=FACE_OUTER_BOUND ( 'NONE', #85839, .T. ) ;
#49804=DIRECTION ( 'NONE',  ( 0.000000000000000000, 0.000000000000000000, 1.000000000000000000 ) ) ;
#49805=FACE_OUTER_BOUND ( 'NONE', #51997, .T. ) ;
#49806=AXIS2_PLACEMENT_3D ( 'NONE', #86250, #76453, #93516 ) ;
#49807=ORIENTED_EDGE ( 'NONE', *, *, #73366, .F. ) ;
#49808=EDGE_CURVE ( 'NONE', #19578, #29149, #62646, .T. ) ;
#49809=CIRCLE ( 'NONE', #53999, 0.1000000000000002554 ) ;
#49810=EDGE_LOOP ( 'NONE', ( #11473, #6070, #16987, #15811 ) ) ;
#49811=CARTESIAN_POINT ( 'NONE',  ( 8.749999999999923617, 2.500000000000000000, 1.372243186433545370 ) ) ;
#49812=VERTEX_POINT ( 'NONE', #104339 ) ;
#49813=CARTESIAN_POINT ( 'NONE',  ( 4.399999999999937295, 2.500000000000000000, 4.576537180435972019 ) ) ;
#49814=EDGE_LOOP ( 'NONE', ( #52707, #78546, #127854, #32440 ) ) ;
#49815=ORIENTED_EDGE ( 'NONE', *, *, #58631, .T. ) ;
#49816=ORIENTED_EDGE ( 'NONE', *, *, #2589, .F. ) ;
#49817=FACE_OUTER_BOUND ( 'NONE', #73827, .T. ) ;
#49818=AXIS2_PLACEMENT_3D ( 'NONE', #73918, #85018, #35296 ) ;
#49819=DIRECTION ( 'NONE',  ( 0.000000000000000000, 0.000000000000000000, -1.000000000000000000 ) ) ;
#49820=DIRECTION ( 'NONE',  ( -0.000000000000000000, -1.000000000000000000, -0.000000000000000000 ) ) ;
#49822=DIRECTION ( 'NONE',  ( 0.000000000000000000, 0.000000000000000000, -1.000000000000000000 ) ) ;
#49823=CARTESIAN_POINT ( 'NONE',  ( -6.250000000000019540, 2.500000000000000000, -2.757883832488654097 ) ) ;
#49824=CARTESIAN_POINT ( 'NONE',  ( 2.899999999999944844, 2.500000000000000000, 3.737306695894644371 ) ) ;
#49826=AXIS2_PLACEMENT_3D ( 'NONE', #87176, #117931, #127133 ) ;
#49827=LINE ( 'NONE', #70737, #100997 ) ;
#49828=DIRECTION ( 'NONE',  ( 0.000000000000000000, 0.000000000000000000, 1.000000000000000000 ) ) ;
#49829=EDGE_LOOP ( 'NONE', ( #108292, #59947 ) ) ;
#49830=VECTOR ( 'NONE', #21500, 1000.000000000000000 ) ;
#49831=ORIENTED_EDGE ( 'NONE', *, *, #23877, .T. ) ;
#49833=LINE ( 'NONE', #70744, #125913 ) ;
#49834=EDGE_LOOP ( 'NONE', ( #66733, #49970 ) ) ;
#49835=VERTEX_POINT ( 'NONE', #104959 ) ;
#49836=DIRECTION ( 'NONE',  ( -0.000000000000000000, -1.000000000000000000, -0.000000000000000000 ) ) ;
#49837=VECTOR ( 'NONE', #96159, 1000.000000000000000 ) ;
#49838=LINE ( 'NONE', #70114, #119368 ) ;
#49839=CONICAL_SURFACE ( 'NONE', #102058, 0.1000000000000000472, 0.003490658503988666988 ) ;
#49840=DIRECTION ( 'NONE',  ( -4.274815082592931898E-19, -0.9999939076577903929, -0.003490651415223739937 ) ) ;
#49842=CARTESIAN_POINT ( 'NONE',  ( -3.100000000000028955, 2.500000000000000000, 4.776537180435972196 ) ) ;
#49843=ORIENTED_EDGE ( 'NONE', *, *, #107776, .T. ) ;
#49844=CIRCLE ( 'NONE', #114663, 0.06509327318403745899 ) ;
#49845=ORIENTED_EDGE ( 'NONE', *, *, #113657, .T. ) ;
#49846=DIRECTION ( 'NONE',  ( 0.000000000000000000, -0.000000000000000000, 1.000000000000000000 ) ) ;
#49847=EDGE_CURVE ( 'NONE', #115142, #55580, #100286, .T. ) ;
#49848=VERTEX_POINT ( 'NONE', #23192 ) ;
#49849=DIRECTION ( 'NONE',  ( 0.000000000000000000, 1.000000000000000000, 0.000000000000000000 ) ) ;
#49850=ORIENTED_EDGE ( 'NONE', *, *, #57066, .T. ) ;
#49851=AXIS2_PLACEMENT_3D ( 'NONE', #98677, #17538, #57488 ) ;
#49852=EDGE_CURVE ( 'NONE', #29412, #41537, #123269, .T. ) ;
#49853=VERTEX_POINT ( 'NONE', #72950 ) ;
#49854=ADVANCED_FACE ( 'NONE', ( #63123 ), #81422, .T. ) ;
#49855=CARTESIAN_POINT ( 'NONE',  ( -3.350000000000028511, 2.500000000000000000, 1.472243186433545459 ) ) ;
#49856=DIRECTION ( 'NONE',  ( 0.000000000000000000, 0.000000000000000000, 1.000000000000000000 ) ) ;
#49857=AXIS2_PLACEMENT_3D ( 'NONE', #38070, #80421, #17771 ) ;
#49858=AXIS2_PLACEMENT_3D ( 'NONE', #28961, #100891, #109441 ) ;
#49859=CARTESIAN_POINT ( 'NONE',  ( -5.000000000000024869, 2.500000000000000000, -5.022947341949754119 ) ) ;
#49860=DIRECTION ( 'NONE',  ( 0.000000000000000000, 1.000000000000000000, 0.000000000000000000 ) ) ;
#49861=EDGE_CURVE ( 'NONE', #87429, #41083, #43874, .T. ) ;
#49862=CARTESIAN_POINT ( 'NONE',  ( -10.60000000000000142, 2.500000000000000000, 4.083716857408421497 ) ) ;
#49863=EDGE_CURVE ( 'NONE', #87369, #66203, #95167, .T. ) ;
#49864=VERTEX_POINT ( 'NONE', #125894 ) ;
#49865=DIRECTION ( 'NONE',  ( 0.000000000000000000, -0.9999939076577903929, 0.003490651415223739937 ) ) ;
#49866=DIRECTION ( 'NONE',  ( 0.000000000000000000, -0.000000000000000000, 1.000000000000000000 ) ) ;
#49867=EDGE_CURVE ( 'NONE', #124699, #54263, #77455, .T. ) ;
#49868=DIRECTION ( 'NONE',  ( -0.000000000000000000, -1.000000000000000000, -0.000000000000000000 ) ) ;
#49869=EDGE_CURVE ( 'NONE', #99646, #36161, #118019, .T. ) ;
#49870=ADVANCED_FACE ( 'NONE', ( #85967 ), #125268, .T. ) ;
#49871=CARTESIAN_POINT ( 'NONE',  ( -3.749999999999991118, 2.500000000000000000, 2.065063509461097624 ) ) ;
#49872=DIRECTION ( 'NONE',  ( 0.000000000000000000, 1.000000000000000000, 0.000000000000000000 ) ) ;
#49873=ORIENTED_EDGE ( 'NONE', *, *, #26028, .F. ) ;
#49874=ORIENTED_EDGE ( 'NONE', *, *, #22119, .T. ) ;
#49875=AXIS2_PLACEMENT_3D ( 'NONE', #33359, #43820, #14318 ) ;
#49876=CARTESIAN_POINT ( 'NONE',  ( 4.999999999999936939, 2.500000000000000000, -0.5928203230275541635 ) ) ;
#49877=EDGE_CURVE ( 'NONE', #127950, #40372, #87656, .T. ) ;
#49878=VERTEX_POINT ( 'NONE', #7410 ) ;
#49879=CARTESIAN_POINT ( 'NONE',  ( 17.28960762337861468, -1.567482926518892761, 5.035524966326045515 ) ) ;
#49880=DIRECTION ( 'NONE',  ( 0.000000000000000000, 0.000000000000000000, 1.000000000000000000 ) ) ;
#49881=AXIS2_PLACEMENT_3D ( 'NONE', #20396, #60336, #100249 ) ;
#49882=AXIS2_PLACEMENT_3D ( 'NONE', #98728, #9721, #67983 ) ;
#49883=VERTEX_POINT ( 'NONE', #17883 ) ;
#49884=CARTESIAN_POINT ( 'NONE',  ( 11.24999999999990763, 12.50000000000000000, -7.188010851410854052 ) ) ;
#49885=CARTESIAN_POINT ( 'NONE',  ( 5.399999999999934630, 2.500000000000000000, -0.6928203230275542523 ) ) ;
#49886=LINE ( 'NONE', #30893, #106803 ) ;
#49887=FACE_OUTER_BOUND ( 'NONE', #102541, .T. ) ;
#49888=AXIS2_PLACEMENT_3D ( 'NONE', #80222, #21960, #60594 ) ;
#49889=CIRCLE ( 'NONE', #54073, 0.09999999999999982514 ) ;
#49890=CONICAL_SURFACE ( 'NONE', #60270, 0.09999999999999982514, 0.003490658503988666988 ) ;
#49891=DIRECTION ( 'NONE',  ( -4.274815082592931898E-19, -0.9999939076577903929, -0.003490651415223739937 ) ) ;
#49892=ORIENTED_EDGE ( 'NONE', *, *, #61117, .F. ) ;
#49893=CARTESIAN_POINT ( 'NONE',  ( 32.15747589919253357, 2.842529944137248243, -4.549402827138433913 ) ) ;
#49894=DIRECTION ( 'NONE',  ( -0.000000000000000000, -1.000000000000000000, -0.000000000000000000 ) ) ;
#49895=CIRCLE ( 'NONE', #62512, 0.06509327318403745899 ) ;
#49896=CARTESIAN_POINT ( 'NONE',  ( 2.499999999999947153, 12.50000000000000000, 0.6928203230275494784 ) ) ;
#49897=CONICAL_SURFACE ( 'NONE', #66597, 0.09999999999999982514, 0.003490658503988666988 ) ;
#49898=ORIENTED_EDGE ( 'NONE', *, *, #106491, .F. ) ;
#49899=CARTESIAN_POINT ( 'NONE',  ( -6.700000000000019718, 2.500000000000000000, 0.09999999999999761857 ) ) ;
#49900=EDGE_CURVE ( 'NONE', #38154, #103846, #18712, .T. ) ;
#49901=ORIENTED_EDGE ( 'NONE', *, *, #91687, .T. ) ;
#49902=EDGE_CURVE ( 'NONE', #34505, #93321, #102349, .T. ) ;
#49903=CARTESIAN_POINT ( 'NONE',  ( -2.500000000000032419, 2.500000000000000000, 0.6928203230275494784 ) ) ;
#49904=CARTESIAN_POINT ( 'NONE',  ( 8.349999999999919709, 12.50000000000000000, 5.802370205355744659 ) ) ;
#49905=CARTESIAN_POINT ( 'NONE',  ( 7.049999999999928768, 12.50000000000000000, 6.495190528383297135 ) ) ;
#49906=EDGE_CURVE ( 'NONE', #7038, #103959, #94021, .T. ) ;
#49907=EDGE_LOOP ( 'NONE', ( #26408, #59256 ) ) ;
#49908=AXIS2_PLACEMENT_3D ( 'NONE', #90156, #18854, #60102 ) ;
#49909=CARTESIAN_POINT ( 'NONE',  ( 12.29999999999990479, 2.500000000000000000, 4.676537180435972552 ) ) ;
#49910=EDGE_CURVE ( 'NONE', #79180, #12963, #28367, .T. ) ;
#49912=AXIS2_PLACEMENT_3D ( 'NONE', #127849, #67627, #97103 ) ;
#49913=AXIS2_PLACEMENT_3D ( 'NONE', #38768, #78679, #79326 ) ;
#49914=EDGE_LOOP ( 'NONE', ( #112964, #110283 ) ) ;
#49915=DIRECTION ( 'NONE',  ( -4.274815082592931898E-19, -0.9999939076577903929, -0.003490651415223739937 ) ) ;
#49916=EDGE_CURVE ( 'NONE', #124473, #4878, #96434, .T. ) ;
#49917=ORIENTED_EDGE ( 'NONE', *, *, #32334, .F. ) ;
#49918=CARTESIAN_POINT ( 'NONE',  ( 9.799999999999913669, 2.500000000000000000, -4.083716857408426826 ) ) ;
#49919=EDGE_CURVE ( 'NONE', #67022, #126753, #35610, .T. ) ;
#49920=EDGE_CURVE ( 'NONE', #50581, #20221, #14485, .T. ) ;
#49921=EDGE_CURVE ( 'NONE', #53157, #79956, #47973, .T. ) ;
#49922=ORIENTED_EDGE ( 'NONE', *, *, #115005, .T. ) ;
#49924=DIRECTION ( 'NONE',  ( 0.000000000000000000, 0.000000000000000000, 1.000000000000000000 ) ) ;
#49925=DIRECTION ( 'NONE',  ( 0.000000000000000000, -0.9999939076577903929, 0.003490651415223739937 ) ) ;
#49926=ORIENTED_EDGE ( 'NONE', *, *, #7040, .F. ) ;
#49927=ORIENTED_EDGE ( 'NONE', *, *, #34382, .F. ) ;
#49928=PLANE ( 'NONE',  #20616 ) ;
#49929=CARTESIAN_POINT ( 'NONE',  ( 8.949999999999921130, 2.500000000000000000, -6.841600689897078702 ) ) ;
#49930=AXIS2_PLACEMENT_3D ( 'NONE', #110818, #31011, #31632 ) ;
#49931=ORIENTED_EDGE ( 'NONE', *, *, #76219, .T. ) ;
#49932=EDGE_CURVE ( 'NONE', #129526, #99163, #115413, .T. ) ;
#49933=CARTESIAN_POINT ( 'NONE',  ( 3.749999999999944045, 2.500000000000000000, -2.857883832488653741 ) ) ;
#49934=DIRECTION ( 'NONE',  ( -0.000000000000000000, 1.000000000000000000, -0.000000000000000000 ) ) ;
#49935=CIRCLE ( 'NONE', #75047, 0.06509327318403745899 ) ;
#49936=CARTESIAN_POINT ( 'NONE',  ( -11.44999999999999751, 2.500000000000000000, 6.048780366869521252 ) ) ;
#49938=DIRECTION ( 'NONE',  ( 0.000000000000000000, 1.000000000000000000, 0.000000000000000000 ) ) ;
#49939=DIRECTION ( 'NONE',  ( -0.000000000000000000, -1.000000000000000000, -0.000000000000000000 ) ) ;
#49940=LINE ( 'NONE', #99671, #90226 ) ;
#49941=CONICAL_SURFACE ( 'NONE', #102246, 0.1000000000000002554, 0.003490658503988666988 ) ;
#49942=ORIENTED_EDGE ( 'NONE', *, *, #58487, .T. ) ;
#49943=ORIENTED_EDGE ( 'NONE', *, *, #42016, .F. ) ;
#49944=AXIS2_PLACEMENT_3D ( 'NONE', #11198, #89768, #40037 ) ;
#49945=AXIS2_PLACEMENT_3D ( 'NONE', #84343, #94159, #114438 ) ;
#49946=ORIENTED_EDGE ( 'NONE', *, *, #53015, .F. ) ;
#49947=ORIENTED_EDGE ( 'NONE', *, *, #98802, .T. ) ;
#49948=CARTESIAN_POINT ( 'NONE',  ( 13.34999999999989662, 2.500000000000000000, -1.372243186433550033 ) ) ;
#49949=CARTESIAN_POINT ( 'NONE',  ( 2.299999999999948752, 2.500000000000000000, -3.883716857408426648 ) ) ;
#49950=CARTESIAN_POINT ( 'NONE',  ( -10.40000000000000213, 12.50000000000000000, -2.276824562219559311E-15 ) ) ;
#49951=AXIS2_PLACEMENT_3D ( 'NONE', #41728, #62005, #61355 ) ;
#49952=EDGE_LOOP ( 'NONE', ( #83437, #27670, #21174, #84290 ) ) ;
#49953=FACE_BOUND ( 'NONE', #125576, .T. ) ;
#49954=EDGE_LOOP ( 'NONE', ( #127975, #128236 ) ) ;
#49955=ADVANCED_FACE ( 'NONE', ( #65698 ), #87262, .T. ) ;
#49956=DIRECTION ( 'NONE',  ( -0.000000000000000000, 1.000000000000000000, -0.000000000000000000 ) ) ;
#49957=DIRECTION ( 'NONE',  ( 0.000000000000000000, 0.000000000000000000, 1.000000000000000000 ) ) ;
#49958=CARTESIAN_POINT ( 'NONE',  ( -1.250000000000036193, 12.50000000000000000, 5.737276932171707422 ) ) ;
#49960=CIRCLE ( 'NONE', #123096, 0.06509327318403745899 ) ;
#49961=CARTESIAN_POINT ( 'NONE',  ( 9.599999999999917932, 2.500000000000000000, -0.6928203230275541413 ) ) ;
#49962=DIRECTION ( 'NONE',  ( 0.000000000000000000, 0.000000000000000000, -1.000000000000000000 ) ) ;
#49963=DIRECTION ( 'NONE',  ( 0.000000000000000000, 1.000000000000000000, 0.000000000000000000 ) ) ;
#49964=CARTESIAN_POINT ( 'NONE',  ( 1.649999999999951950, 12.50000000000000000, -5.802370205355749988 ) ) ;
#49965=CARTESIAN_POINT ( 'NONE',  ( -4.150000000000024336, 12.50000000000000000, -2.230156782645139391 ) ) ;
#49966=CARTESIAN_POINT ( 'NONE',  ( 6.899999999999926636, 12.50000000000000000, -0.4115034346978156399 ) ) ;
#49967=ORIENTED_EDGE ( 'NONE', *, *, #63331, .T. ) ;
#49968=ORIENTED_EDGE ( 'NONE', *, *, #103325, .F. ) ;
#49969=EDGE_CURVE ( 'NONE', #12970, #128176, #16578, .T. ) ;
#49970=ORIENTED_EDGE ( 'NONE', *, *, #86935, .T. ) ;
#49972=DIRECTION ( 'NONE',  ( 0.000000000000000000, 1.000000000000000000, 0.000000000000000000 ) ) ;
#49973=AXIS2_PLACEMENT_3D ( 'NONE', #67940, #88201, #18193 ) ;
#49974=DIRECTION ( 'NONE',  ( -0.000000000000000000, 1.000000000000000000, -0.000000000000000000 ) ) ;
#49975=VERTEX_POINT ( 'NONE', #55875 ) ;
#49976=ORIENTED_EDGE ( 'NONE', *, *, #107799, .F. ) ;
#49977=ORIENTED_EDGE ( 'NONE', *, *, #54792, .F. ) ;
#49978=DIRECTION ( 'NONE',  ( 0.000000000000000000, 1.000000000000000000, 0.000000000000000000 ) ) ;
#49979=AXIS2_PLACEMENT_3D ( 'NONE', #8462, #47771, #87673 ) ;
#49980=AXIS2_PLACEMENT_3D ( 'NONE', #29083, #21168, #123085 ) ;
#49981=DIRECTION ( 'NONE',  ( 0.000000000000000000, -0.000000000000000000, 1.000000000000000000 ) ) ;
#49982=CARTESIAN_POINT ( 'NONE',  ( -5.600000000000020073, 2.500000000000000000, 3.983716857408420964 ) ) ;
#49983=CARTESIAN_POINT ( 'NONE',  ( 3.149999999999942624, 2.500000000000000000, 6.841600689897072485 ) ) ;
#49984=DIRECTION ( 'NONE',  ( -0.000000000000000000, -1.000000000000000000, -0.000000000000000000 ) ) ;
#49985=DIRECTION ( 'NONE',  ( 0.000000000000000000, -0.9999939076577903929, 0.003490651415223739937 ) ) ;
#49986=CARTESIAN_POINT ( 'NONE',  ( -4.550000000000022915, 12.50000000000000000, 2.230156782645134950 ) ) ;
#49987=ADVANCED_FACE ( 'NONE', ( #27698 ), #127844, .T. ) ;
#49988=ORIENTED_EDGE ( 'NONE', *, *, #117380, .F. ) ;
#49989=VECTOR ( 'NONE', #80416, 1000.000000000000000 ) ;
#49990=FACE_OUTER_BOUND ( 'NONE', #114980, .T. ) ;
#49991=EDGE_LOOP ( 'NONE', ( #45687, #89952, #102819, #128535 ) ) ;
#49992=CONICAL_SURFACE ( 'NONE', #66671, 0.1000000000000002554, 0.003490658503988666988 ) ;
#49993=ORIENTED_EDGE ( 'NONE', *, *, #93965, .F. ) ;
#49994=VERTEX_POINT ( 'NONE', #10007 ) ;
#49995=CARTESIAN_POINT ( 'NONE',  ( -0.4000000000000331624, 2.500000000000000000, -0.5928203230275518321 ) ) ;
#49996=ORIENTED_EDGE ( 'NONE', *, *, #5934, .T. ) ;
#49997=EDGE_LOOP ( 'NONE', ( #45557, #98634, #75104, #66501 ) ) ;
#49998=AXIS2_PLACEMENT_3D ( 'NONE', #66941, #68889, #76140 ) ;
#49999=DIRECTION ( 'NONE',  ( -0.000000000000000000, -1.000000000000000000, -0.000000000000000000 ) ) ;
#50000=CIRCLE ( 'NONE', #31208, 0.09999999999999982514 ) ;
#50001=CARTESIAN_POINT ( 'NONE',  ( 0.5999999999999621192, 12.50000000000000000, 0.4115034346978132529 ) ) ;
#50002=PLANE ( 'NONE',  #77104 ) ;
#50003=CARTESIAN_POINT ( 'NONE',  ( -14.34999999999998543, 2.500000000000000000, 2.511473670974877503 ) ) ;
#50004=CARTESIAN_POINT ( 'NONE',  ( 2.049999999999950084, 2.500000000000000000, -2.165063509461101710 ) ) ;
#50006=CARTESIAN_POINT ( 'NONE',  ( 14.19999999999989626, 12.50000000000000000, -2.276824562219559311E-15 ) ) ;
#50007=AXIS2_PLACEMENT_3D ( 'NONE', #48667, #79425, #69582 ) ;
#50008=ORIENTED_EDGE ( 'NONE', *, *, #11037, .F. ) ;
#50009=CARTESIAN_POINT ( 'NONE',  ( 7.949999999999925571, 2.500000000000000000, -6.495190528383302464 ) ) ;
#50010=EDGE_CURVE ( 'NONE', #31018, #64039, #119068, .T. ) ;
#50011=ORIENTED_EDGE ( 'NONE', *, *, #118658, .T. ) ;
#50013=CARTESIAN_POINT ( 'NONE',  ( 3.749999999999940492, 12.50000000000000000, 2.857883832488649301 ) ) ;
#50014=CONICAL_SURFACE ( 'NONE', #68852, 0.1000000000000000472, 0.003490658503988666988 ) ;
#50015=ORIENTED_EDGE ( 'NONE', *, *, #34649, .F. ) ;
#50016=DIRECTION ( 'NONE',  ( 0.000000000000000000, 0.000000000000000000, 1.000000000000000000 ) ) ;
#50017=CARTESIAN_POINT ( 'NONE',  ( -11.84999999999999787, 2.500000000000000000, -6.941600689897074794 ) ) ;
#50018=EDGE_LOOP ( 'NONE', ( #71050, #47748, #7435, #120621 ) ) ;
#50019=EDGE_CURVE ( 'NONE', #82469, #54523, #64681, .T. ) ;
#50020=CONICAL_SURFACE ( 'NONE', #70822, 0.09999999999999982514, 0.003490658503988666988 ) ;
#50021=CARTESIAN_POINT ( 'NONE',  ( 3.149999999999944400, 12.50000000000000000, 1.818653347947321475 ) ) ;
#50022=EDGE_LOOP ( 'NONE', ( #25137, #88712 ) ) ;
#50023=EDGE_CURVE ( 'NONE', #116662, #104656, #31585, .T. ) ;
#50024=EDGE_CURVE ( 'NONE', #41483, #39986, #50131, .T. ) ;
#50025=EDGE_LOOP ( 'NONE', ( #68759, #30098, #126817, #3944 ) ) ;
#50026=FACE_OUTER_BOUND ( 'NONE', #112747, .T. ) ;
#50027=DIRECTION ( 'NONE',  ( 0.000000000000000000, 0.000000000000000000, -1.000000000000000000 ) ) ;
#50028=EDGE_CURVE ( 'NONE', #85332, #24109, #125329, .T. ) ;
#50031=CARTESIAN_POINT ( 'NONE',  ( -13.09999999999999254, 2.500000000000000000, 0.2464101615137777868 ) ) ;
#50032=CIRCLE ( 'NONE', #39658, 0.1000000000000000472 ) ;
#50033=VECTOR ( 'NONE', #54066, 1000.000000000000000 ) ;
#50034=DIRECTION ( 'NONE',  ( -0.000000000000000000, 1.000000000000000000, -0.000000000000000000 ) ) ;
#50035=ORIENTED_EDGE ( 'NONE', *, *, #43687, .F. ) ;
#50036=DIRECTION ( 'NONE',  ( 0.000000000000000000, -0.9999939076577903929, 0.003490651415223739937 ) ) ;
#50037=VECTOR ( 'NONE', #101150, 1000.000000000000000 ) ;
#50038=EDGE_CURVE ( 'NONE', #49975, #28873, #41721, .T. ) ;
#50039=VERTEX_POINT ( 'NONE', #69560 ) ;
#50040=EDGE_CURVE ( 'NONE', #7340, #63939, #83575, .T. ) ;
#50041=CARTESIAN_POINT ( 'NONE',  ( -13.09999999999999254, 2.500000000000000000, -0.4464101615137741064 ) ) ;
#50042=DIRECTION ( 'NONE',  ( 0.000000000000000000, 1.000000000000000000, 0.000000000000000000 ) ) ;
#50043=ADVANCED_FACE ( 'NONE', ( #8690 ), #4118, .T. ) ;
#50044=AXIS2_PLACEMENT_3D ( 'NONE', #117641, #115726, #48289 ) ;
#50045=VECTOR ( 'NONE', #82122, 1000.000000000000000 ) ;
#50048=PLANE ( 'NONE',  #67732 ) ;
#50049=PLANE ( 'NONE',  #86163 ) ;
#50050=CARTESIAN_POINT ( 'NONE',  ( -1.650000000000034328, 12.50000000000000000, -2.230156782645139391 ) ) ;
#50051=CARTESIAN_POINT ( 'NONE',  ( -1.650000000000034772, 2.500000000000000000, 5.802370205355744659 ) ) ;
#50052=ORIENTED_EDGE ( 'NONE', *, *, #51958, .F. ) ;
#50053=AXIS2_PLACEMENT_3D ( 'NONE', #129545, #60155, #10384 ) ;
#50055=FACE_OUTER_BOUND ( 'NONE', #107838, .T. ) ;
#50056=FACE_OUTER_BOUND ( 'NONE', #44309, .T. ) ;
#50057=DIRECTION ( 'NONE',  ( 0.000000000000000000, 1.000000000000000000, 0.000000000000000000 ) ) ;
#50058=ORIENTED_EDGE ( 'NONE', *, *, #12560, .F. ) ;
#50059=DIRECTION ( 'NONE',  ( 0.000000000000000000, 0.000000000000000000, -1.000000000000000000 ) ) ;
#50060=VERTEX_POINT ( 'NONE', #119304 ) ;
#50061=ORIENTED_EDGE ( 'NONE', *, *, #101964, .T. ) ;
#50062=CARTESIAN_POINT ( 'NONE',  ( -3.950000000000029932, 2.500000000000000000, -6.148780366869526226 ) ) ;
#50063=VECTOR ( 'NONE', #18531, 1000.000000000000000 ) ;
#50064=ORIENTED_EDGE ( 'NONE', *, *, #100968, .T. ) ;
#50065=DIRECTION ( 'NONE',  ( -0.000000000000000000, -1.000000000000000000, -0.000000000000000000 ) ) ;
#50066=DIRECTION ( 'NONE',  ( 0.000000000000000000, 0.000000000000000000, 1.000000000000000000 ) ) ;
#50068=AXIS2_PLACEMENT_3D ( 'NONE', #84945, #124882, #25367 ) ;
#50069=CARTESIAN_POINT ( 'NONE',  ( 10.64999999999991331, 12.50000000000000000, 6.776507416713035248 ) ) ;
#50070=DIRECTION ( 'NONE',  ( -0.000000000000000000, -1.000000000000000000, -0.000000000000000000 ) ) ;
#50071=FACE_OUTER_BOUND ( 'NONE', #45069, .T. ) ;
#50072=EDGE_CURVE ( 'NONE', #35674, #9000, #60599, .T. ) ;
#50073=CIRCLE ( 'NONE', #119001, 0.06509327318403745899 ) ;
#50074=ORIENTED_EDGE ( 'NONE', *, *, #101011, .T. ) ;
#50075=CIRCLE ( 'NONE', #4073, 0.06509327318403745899 ) ;
#50077=CIRCLE ( 'NONE', #83518, 0.06509327318403745899 ) ;
#50078=VERTEX_POINT ( 'NONE', #119963 ) ;
#50079=EDGE_CURVE ( 'NONE', #103728, #91651, #78768, .T. ) ;
#50080=ORIENTED_EDGE ( 'NONE', *, *, #36483, .T. ) ;
#50081=DIRECTION ( 'NONE',  ( 0.000000000000000000, 0.000000000000000000, 1.000000000000000000 ) ) ;
#50082=DIRECTION ( 'NONE',  ( -0.000000000000000000, -1.000000000000000000, -0.000000000000000000 ) ) ;
#50083=CARTESIAN_POINT ( 'NONE',  ( 2.499999999999947153, 2.500000000000000000, 0.6928203230275494784 ) ) ;
#50084=FACE_BOUND ( 'NONE', #23913, .T. ) ;
#50085=ORIENTED_EDGE ( 'NONE', *, *, #95342, .F. ) ;
#50086=AXIS2_PLACEMENT_3D ( 'NONE', #92390, #24951, #24308 ) ;
#50087=CARTESIAN_POINT ( 'NONE',  ( -14.34999999999998543, 12.50000000000000000, -1.818653347947323695 ) ) ;
#50088=CARTESIAN_POINT ( 'NONE',  ( 11.64999999999990266, 12.50000000000000000, 2.165063509461097713 ) ) ;
#50090=EDGE_CURVE ( 'NONE', #98576, #94293, #83293, .T. ) ;
#50091=CONICAL_SURFACE ( 'NONE', #10351, 0.1000000000000002554, 0.003490658503988666988 ) ;
#50092=DIRECTION ( 'NONE',  ( 0.000000000000000000, 1.000000000000000000, 0.000000000000000000 ) ) ;
#50093=CARTESIAN_POINT ( 'NONE',  ( -13.34999999999999076, 2.500000000000000000, -1.372243186433547812 ) ) ;
#50094=CARTESIAN_POINT ( 'NONE',  ( -10.00000000000000533, 2.500000000000000000, 0.7928203230275495672 ) ) ;
#50095=CARTESIAN_POINT ( 'NONE',  ( -6.650000000000014566, 2.500000000000000000, 1.572243186433545548 ) ) ;
#50096=FACE_OUTER_BOUND ( 'NONE', #111601, .T. ) ;
#50097=CARTESIAN_POINT ( 'NONE',  ( 1.849999999999951017, 2.500000000000000000, -6.248780366869526759 ) ) ;
#50098=DIRECTION ( 'NONE',  ( 0.000000000000000000, 0.000000000000000000, 1.000000000000000000 ) ) ;
#50099=ORIENTED_EDGE ( 'NONE', *, *, #97849, .F. ) ;
#50100=VERTEX_POINT ( 'NONE', #68918 ) ;
#50101=EDGE_LOOP ( 'NONE', ( #32855, #23230, #11646, #69496 ) ) ;
#50102=VERTEX_POINT ( 'NONE', #108835 ) ;
#50103=LINE ( 'NONE', #52023, #37009 ) ;
#50104=CARTESIAN_POINT ( 'NONE',  ( -5.400000000000024336, 2.500000000000000000, -3.637306695894650055 ) ) ;
#50105=ORIENTED_EDGE ( 'NONE', *, *, #126160, .F. ) ;
#50106=FACE_BOUND ( 'NONE', #122501, .T. ) ;
#50107=EDGE_CURVE ( 'NONE', #74504, #88669, #129166, .T. ) ;
#50108=DIRECTION ( 'NONE',  ( 0.000000000000000000, 1.000000000000000000, 0.000000000000000000 ) ) ;
#50109=FACE_OUTER_BOUND ( 'NONE', #8761, .T. ) ;
#50110=CARTESIAN_POINT ( 'NONE',  ( 1.449999999999951328, 2.500000000000000000, 2.511473670974873507 ) ) ;
#50111=DIRECTION ( 'NONE',  ( 0.000000000000000000, 0.000000000000000000, 1.000000000000000000 ) ) ;
#50112=CARTESIAN_POINT ( 'NONE',  ( 3.149999999999942624, 2.500000000000000000, 6.248780366869521430 ) ) ;
#50113=LINE ( 'NONE', #128687, #124950 ) ;
#50114=EDGE_LOOP ( 'NONE', ( #95492, #91559 ) ) ;
#50115=EDGE_LOOP ( 'NONE', ( #7804, #39267 ) ) ;
#50116=ORIENTED_EDGE ( 'NONE', *, *, #61739, .F. ) ;
#50118=ADVANCED_FACE ( 'NONE', ( #51243 ), #19155, .T. ) ;
#50119=ORIENTED_EDGE ( 'NONE', *, *, #49916, .T. ) ;
#50120=EDGE_LOOP ( 'NONE', ( #50772, #30017, #26765, #12196 ) ) ;
#50121=DIRECTION ( 'NONE',  ( -0.000000000000000000, 1.000000000000000000, -0.000000000000000000 ) ) ;
#50122=FACE_OUTER_BOUND ( 'NONE', #65732, .T. ) ;
#50123=VECTOR ( 'NONE', #104050, 1000.000000000000000 ) ;
#50124=ORIENTED_EDGE ( 'NONE', *, *, #24864, .F. ) ;
#50125=PLANE ( 'NONE',  #99932 ) ;
#50126=AXIS2_PLACEMENT_3D ( 'NONE', #8149, #36982, #27790 ) ;
#50127=CARTESIAN_POINT ( 'NONE',  ( 13.34999999999989662, 12.50000000000000000, -2.857883832488653741 ) ) ;
#50129=DIRECTION ( 'NONE',  ( 0.000000000000000000, 1.000000000000000000, 0.000000000000000000 ) ) ;
#50130=CARTESIAN_POINT ( 'NONE',  ( -0.4000000000000401013, 2.500000000000000000, -3.537306695894649966 ) ) ;
#50131=CIRCLE ( 'NONE', #127479, 0.06509327318403741736 ) ;
#50132=EDGE_CURVE ( 'NONE', #38338, #105257, #56162, .T. ) ;
#50133=ORIENTED_EDGE ( 'NONE', *, *, #38479, .T. ) ;
#50134=DIRECTION ( 'NONE',  ( 0.000000000000000000, 0.000000000000000000, 1.000000000000000000 ) ) ;
#50135=VECTOR ( 'NONE', #59855, 1000.000000000000000 ) ;
#50136=ORIENTED_EDGE ( 'NONE', *, *, #126969, .T. ) ;
#50137=VERTEX_POINT ( 'NONE', #60420 ) ;
#50138=CARTESIAN_POINT ( 'NONE',  ( -14.34999999999998543, 2.500000000000000000, 1.818653347947325472 ) ) ;
#50139=CARTESIAN_POINT ( 'NONE',  ( -6.850000000000013856, 12.50000000000000000, 2.511473670974873507 ) ) ;
#50140=CARTESIAN_POINT ( 'NONE',  ( -10.60000000000000320, 12.50000000000000000, -4.676537180435973440 ) ) ;
#50141=EDGE_CURVE ( 'NONE', #94650, #109859, #74961, .T. ) ;
#50142=VERTEX_POINT ( 'NONE', #13210 ) ;
#50144=CARTESIAN_POINT ( 'NONE',  ( -9.150000000000009237, 12.50000000000000000, 2.165063509461097713 ) ) ;
#50145=FACE_OUTER_BOUND ( 'NONE', #90644, .T. ) ;
#50147=DIRECTION ( 'NONE',  ( 0.000000000000000000, 0.000000000000000000, 1.000000000000000000 ) ) ;
#50148=ORIENTED_EDGE ( 'NONE', *, *, #18343, .T. ) ;
#50149=DIRECTION ( 'NONE',  ( 0.000000000000000000, -0.9999939076577903929, 0.003490651415223739937 ) ) ;
#50150=ORIENTED_EDGE ( 'NONE', *, *, #14023, .T. ) ;
#50151=CARTESIAN_POINT ( 'NONE',  ( 16.55874544816221317, -0.4845305829210151960, -6.091953208799018249 ) ) ;
#50152=CIRCLE ( 'NONE', #37629, 0.06509327318403745899 ) ;
#50153=VECTOR ( 'NONE', #558, 1000.000000000000000 ) ;
#50154=VERTEX_POINT ( 'NONE', #63626 ) ;
#50156=ADVANCED_FACE ( 'NONE', ( #21770 ), #16445, .T. ) ;
#50157=CARTESIAN_POINT ( 'NONE',  ( 59.86275542849503495, -3.775834014907373248, 4.995382520279711080 ) ) ;
#50158=DIRECTION ( 'NONE',  ( 0.000000000000000000, -0.9999939076577903929, 0.003490651415223739937 ) ) ;
#50159=CARTESIAN_POINT ( 'NONE',  ( 12.09999999999990550, 2.500000000000000000, 3.737306695894644371 ) ) ;
#50160=VERTEX_POINT ( 'NONE', #11929 ) ;
#50161=AXIS2_PLACEMENT_3D ( 'NONE', #17951, #45497, #26494 ) ;
#50162=EDGE_CURVE ( 'NONE', #10500, #47021, #64489, .T. ) ;
#50163=CARTESIAN_POINT ( 'NONE',  ( 4.399999999999937295, 12.50000000000000000, 4.676537180435972552 ) ) ;
#50164=DIRECTION ( 'NONE',  ( 0.000000000000000000, 0.000000000000000000, 1.000000000000000000 ) ) ;
#50165=EDGE_LOOP ( 'NONE', ( #99608, #70746 ) ) ;
#50166=EDGE_LOOP ( 'NONE', ( #70410, #75465, #9719, #27549 ) ) ;
#50167=EDGE_CURVE ( 'NONE', #111265, #91437, #31346, .T. ) ;
#50168=EDGE_CURVE ( 'NONE', #90001, #111704, #18519, .T. ) ;
#50169=ORIENTED_EDGE ( 'NONE', *, *, #119651, .F. ) ;
#50170=DIRECTION ( 'NONE',  ( 0.000000000000000000, 0.000000000000000000, 1.000000000000000000 ) ) ;
#50171=CARTESIAN_POINT ( 'NONE',  ( -0.8500000000000386136, 2.500000000000000000, 5.802370205355744659 ) ) ;
#50172=CARTESIAN_POINT ( 'NONE',  ( -10.84999999999999964, 2.500000000000000000, 2.757883832488649656 ) ) ;
#50173=EDGE_CURVE ( 'NONE', #63537, #12708, #102154, .T. ) ;
#50175=AXIS2_PLACEMENT_3D ( 'NONE', #29611, #51204, #70824 ) ;
#50176=EDGE_CURVE ( 'NONE', #70566, #83042, #89629, .T. ) ;
#50177=CARTESIAN_POINT ( 'NONE',  ( -0.2000000000000408673, 2.500000000000000000, -3.983716857408426293 ) ) ;
#50178=DIRECTION ( 'NONE',  ( 0.000000000000000000, 1.000000000000000000, 0.000000000000000000 ) ) ;
#50179=VECTOR ( 'NONE', #30266, 1000.000000000000000 ) ;
#50180=DIRECTION ( 'NONE',  ( 0.000000000000000000, -0.000000000000000000, 1.000000000000000000 ) ) ;
#50181=FACE_OUTER_BOUND ( 'NONE', #122342, .T. ) ;
#50182=DIRECTION ( 'NONE',  ( -0.000000000000000000, -1.000000000000000000, -0.000000000000000000 ) ) ;
#50184=EDGE_CURVE ( 'NONE', #51769, #79731, #83269, .T. ) ;
#50185=CIRCLE ( 'NONE', #110797, 0.06509327318403745899 ) ;
#50187=ADVANCED_FACE ( 'NONE', ( #22426 ), #43989, .T. ) ;
#50188=ADVANCED_FACE ( 'NONE', ( #93092 ), #51986, .T. ) ;
#50189=EDGE_LOOP ( 'NONE', ( #41371, #52220, #86403, #23848 ) ) ;
#50190=VECTOR ( 'NONE', #48448, 1000.000000000000000 ) ;
#50191=DIRECTION ( 'NONE',  ( 0.000000000000000000, -0.9999939076577903929, 0.003490651415223739937 ) ) ;
#50192=FACE_OUTER_BOUND ( 'NONE', #34840, .T. ) ;
#50193=CARTESIAN_POINT ( 'NONE',  ( -12.49999999999999289, 12.50000000000000000, 3.572213422710607489 ) ) ;
#50194=LINE ( 'NONE', #41666, #52640 ) ;
#50195=CARTESIAN_POINT ( 'NONE',  ( -6.450000000000014388, 2.500000000000000000, 6.248780366869521430 ) ) ;
#50196=EDGE_CURVE ( 'NONE', #46534, #83081, #49844, .T. ) ;
#50197=ORIENTED_EDGE ( 'NONE', *, *, #104485, .F. ) ;
#50198=DIRECTION ( 'NONE',  ( 0.000000000000000000, 0.000000000000000000, 1.000000000000000000 ) ) ;
#50199=PLANE ( 'NONE',  #40766 ) ;
#50200=DIRECTION ( 'NONE',  ( -0.000000000000000000, 1.000000000000000000, -0.000000000000000000 ) ) ;
#50201=ORIENTED_EDGE ( 'NONE', *, *, #120026, .T. ) ;
#50203=EDGE_LOOP ( 'NONE', ( #19186, #92945, #127463, #8083 ) ) ;
#50204=PLANE ( 'NONE',  #703 ) ;
#50205=VERTEX_POINT ( 'NONE', #82628 ) ;
#50206=ORIENTED_EDGE ( 'NONE', *, *, #60251, .F. ) ;
#50207=CARTESIAN_POINT ( 'NONE',  ( 3.099999999999945022, 2.500000000000000000, -0.4464101615137783252 ) ) ;
#50208=CARTESIAN_POINT ( 'NONE',  ( 20.06694580393876137, 2.635910463901537160, -2.269534205243695091 ) ) ;
#50209=DIRECTION ( 'NONE',  ( 0.000000000000000000, 0.000000000000000000, -1.000000000000000000 ) ) ;
#50210=CARTESIAN_POINT ( 'NONE',  ( 14.59999999999989484, 12.50000000000000000, 0.7579135962115869374 ) ) ;
#50211=VERTEX_POINT ( 'NONE', #112078 ) ;
#50213=CONICAL_SURFACE ( 'NONE', #98303, 0.1000000000000002554, 0.003490658503988666988 ) ;
#50214=CARTESIAN_POINT ( 'NONE',  ( 11.89999999999990443, 2.500000000000000000, 0.4464101615137736623 ) ) ;
#50215=ORIENTED_EDGE ( 'NONE', *, *, #84906, .T. ) ;
#50216=FACE_OUTER_BOUND ( 'NONE', #48994, .T. ) ;
#50217=DIRECTION ( 'NONE',  ( -4.274815082592931898E-19, -0.9999939076577903929, -0.003490651415223739937 ) ) ;
#50218=LINE ( 'NONE', #88165, #127006 ) ;
#50219=ORIENTED_EDGE ( 'NONE', *, *, #55304, .F. ) ;
#50220=AXIS2_PLACEMENT_3D ( 'NONE', #25689, #35532, #87178 ) ;
#50221=EDGE_CURVE ( 'NONE', #125995, #117711, #58021, .T. ) ;
#50222=EDGE_LOOP ( 'NONE', ( #13389, #111835, #92422, #62580 ) ) ;
#50223=ORIENTED_EDGE ( 'NONE', *, *, #2219, .T. ) ;
#50224=EDGE_LOOP ( 'NONE', ( #414, #44326 ) ) ;
#50225=ADVANCED_FACE ( 'NONE', ( #104183 ), #32889, .T. ) ;
#50226=ORIENTED_EDGE ( 'NONE', *, *, #39538, .F. ) ;
#50227=CARTESIAN_POINT ( 'NONE',  ( 6.449999999999930012, 12.50000000000000000, 1.883746621131358934 ) ) ;
#50228=CARTESIAN_POINT ( 'NONE',  ( 10.89704209839426419, 1.499999999999809708, 8.980393934824158819 ) ) ;
#50229=CARTESIAN_POINT ( 'NONE',  ( -9.350000000000006750, 2.500000000000000000, 2.511473670974873507 ) ) ;
#50230=FACE_BOUND ( 'NONE', #2177, .T. ) ;
#50231=DIRECTION ( 'NONE',  ( -0.000000000000000000, 1.000000000000000000, -0.000000000000000000 ) ) ;
#50233=DIRECTION ( 'NONE',  ( 0.000000000000000000, 0.000000000000000000, 1.000000000000000000 ) ) ;
#50234=DIRECTION ( 'NONE',  ( -0.000000000000000000, 1.000000000000000000, -0.000000000000000000 ) ) ;
#50235=CARTESIAN_POINT ( 'NONE',  ( -14.79999999999998472, 12.50000000000000000, 0.3464101615137758494 ) ) ;
#50237=DIRECTION ( 'NONE',  ( 0.000000000000000000, 0.000000000000000000, 1.000000000000000000 ) ) ;
#50238=CIRCLE ( 'NONE', #81533, 0.06509327318403745899 ) ;
#50239=CONICAL_SURFACE ( 'NONE', #64799, 0.1000000000000000472, 0.003490658503988666988 ) ;
#50240=DIRECTION ( 'NONE',  ( 0.000000000000000000, 1.000000000000000000, 0.000000000000000000 ) ) ;
#50241=ORIENTED_EDGE ( 'NONE', *, *, #85583, .T. ) ;
#50242=VERTEX_POINT ( 'NONE', #94353 ) ;
#50243=ORIENTED_EDGE ( 'NONE', *, *, #4766, .F. ) ;
#50244=ORIENTED_EDGE ( 'NONE', *, *, #107469, .F. ) ;
#50245=DIRECTION ( 'NONE',  ( -0.000000000000000000, 1.000000000000000000, -0.000000000000000000 ) ) ;
#50246=CARTESIAN_POINT ( 'NONE',  ( 12.09999999999990550, 2.500000000000000000, -3.637306695894650055 ) ) ;
#50247=FACE_BOUND ( 'NONE', #49954, .T. ) ;
#50248=LINE ( 'NONE', #39796, #54038 ) ;
#50249=VERTEX_POINT ( 'NONE', #62971 ) ;
#50250=FACE_OUTER_BOUND ( 'NONE', #77382, .T. ) ;
#50251=CARTESIAN_POINT ( 'NONE',  ( -13.29999999999999005, 2.500000000000000000, -4.230127018922199333 ) ) ;
#50252=CARTESIAN_POINT ( 'NONE',  ( -6.050000000000022027, 2.500000000000000000, -6.148780366869526226 ) ) ;
#50253=CARTESIAN_POINT ( 'NONE',  ( 7.499999999999961808, 2.500000000000000000, 4.430127018922196847 ) ) ;
#50254=CIRCLE ( 'NONE', #119205, 0.06509327318403745899 ) ;
#50255=ORIENTED_EDGE ( 'NONE', *, *, #99513, .T. ) ;
#50256=DIRECTION ( 'NONE',  ( 0.000000000000000000, 0.000000000000000000, 1.000000000000000000 ) ) ;
#50257=CONICAL_SURFACE ( 'NONE', #56493, 0.1000000000000002554, 0.003490658503988666988 ) ;
#50258=ADVANCED_FACE ( 'NONE', ( #4663 ), #33214, .T. ) ;
#50260=ORIENTED_EDGE ( 'NONE', *, *, #2365, .F. ) ;
#50261=DIRECTION ( 'NONE',  ( 0.000000000000000000, 0.000000000000000000, -1.000000000000000000 ) ) ;
#50262=CARTESIAN_POINT ( 'NONE',  ( 5.399999999999931966, 2.500000000000000000, 4.330127018922196314 ) ) ;
#50263=ORIENTED_EDGE ( 'NONE', *, *, #88559, .T. ) ;
#50265=DIRECTION ( 'NONE',  ( -0.000000000000000000, -1.000000000000000000, -0.000000000000000000 ) ) ;
#50266=DIRECTION ( 'NONE',  ( 0.000000000000000000, -0.000000000000000000, 1.000000000000000000 ) ) ;
#50267=VECTOR ( 'NONE', #96573, 1000.000000000000000 ) ;
#50269=EDGE_CURVE ( 'NONE', #15198, #7354, #8046, .T. ) ;
#50270=EDGE_CURVE ( 'NONE', #100839, #59702, #26914, .T. ) ;
#50271=DIRECTION ( 'NONE',  ( 0.000000000000000000, 1.000000000000000000, 0.000000000000000000 ) ) ;
#50272=EDGE_LOOP ( 'NONE', ( #122410, #20423, #6362, #102612 ) ) ;
#50273=DIRECTION ( 'NONE',  ( 0.000000000000000000, 0.000000000000000000, -1.000000000000000000 ) ) ;
#50274=ORIENTED_EDGE ( 'NONE', *, *, #3963, .T. ) ;
#50276=EDGE_LOOP ( 'NONE', ( #47758, #111883, #29131, #41738 ) ) ;
#50277=FACE_OUTER_BOUND ( 'NONE', #77551, .T. ) ;
#50278=DIRECTION ( 'NONE',  ( 0.000000000000000000, 0.000000000000000000, 1.000000000000000000 ) ) ;
#50279=DIRECTION ( 'NONE',  ( 0.000000000000000000, 0.000000000000000000, 1.000000000000000000 ) ) ;
#50280=DIRECTION ( 'NONE',  ( -0.000000000000000000, -1.000000000000000000, -0.000000000000000000 ) ) ;
#50281=EDGE_CURVE ( 'NONE', #91248, #60649, #10118, .T. ) ;
#50282=DIRECTION ( 'NONE',  ( 0.000000000000000000, -0.000000000000000000, 1.000000000000000000 ) ) ;
#50283=VERTEX_POINT ( 'NONE', #66182 ) ;
#50284=ORIENTED_EDGE ( 'NONE', *, *, #84438, .T. ) ;
#50285=ORIENTED_EDGE ( 'NONE', *, *, #53423, .T. ) ;
#50286=DIRECTION ( 'NONE',  ( -0.000000000000000000, 1.000000000000000000, -0.000000000000000000 ) ) ;
#50288=AXIS2_PLACEMENT_3D ( 'NONE', #57378, #9567, #108402 ) ;
#50289=DIRECTION ( 'NONE',  ( -0.000000000000000000, 1.000000000000000000, -0.000000000000000000 ) ) ;
#50290=ORIENTED_EDGE ( 'NONE', *, *, #106888, .F. ) ;
#50291=VERTEX_POINT ( 'NONE', #36750 ) ;
#50292=ORIENTED_EDGE ( 'NONE', *, *, #116237, .F. ) ;
#50293=AXIS2_PLACEMENT_3D ( 'NONE', #90851, #102594, #2449 ) ;
#50294=DIRECTION ( 'NONE',  ( 0.000000000000000000, 0.000000000000000000, -1.000000000000000000 ) ) ;
#50295=EDGE_LOOP ( 'NONE', ( #90470, #44736, #60897, #31294 ) ) ;
#50296=CARTESIAN_POINT ( 'NONE',  ( 12.89999999999989910, 12.50000000000000000, -0.6928203230275542523 ) ) ;
#50297=CIRCLE ( 'NONE', #41981, 0.06509327318403745899 ) ;
#50298=CARTESIAN_POINT ( 'NONE',  ( -4.400000000000028777, 12.50000000000000000, -3.983716857408426293 ) ) ;
#50299=CARTESIAN_POINT ( 'NONE',  ( -6.650000000000014566, 12.50000000000000000, 1.472243186433545459 ) ) ;
#50300=LINE ( 'NONE', #9729, #69578 ) ;
#50301=DIRECTION ( 'NONE',  ( 0.000000000000000000, 0.000000000000000000, 1.000000000000000000 ) ) ;
#50302=CARTESIAN_POINT ( 'NONE',  ( -4.800000000000022915, 2.500000000000000000, 3.983716857408420076 ) ) ;
#50303=CARTESIAN_POINT ( 'NONE',  ( -12.94999999999999218, 2.500000000000000000, 2.165063509461101265 ) ) ;
#50304=EDGE_LOOP ( 'NONE', ( #10288, #108403 ) ) ;
#50305=ORIENTED_EDGE ( 'NONE', *, *, #14693, .T. ) ;
#50306=EDGE_CURVE ( 'NONE', #46758, #97470, #106350, .T. ) ;
#50307=PLANE ( 'NONE',  #59116 ) ;
#50308=ORIENTED_EDGE ( 'NONE', *, *, #34059, .F. ) ;
#50309=ORIENTED_EDGE ( 'NONE', *, *, #65818, .F. ) ;
#50310=ADVANCED_FACE ( 'NONE', ( #105477 ), #45724, .T. ) ;
#50311=DIRECTION ( 'NONE',  ( 0.000000000000000000, 1.000000000000000000, 0.000000000000000000 ) ) ;
#50312=CARTESIAN_POINT ( 'NONE',  ( -2.900000000000029665, 12.50000000000000000, 4.330127018922196314 ) ) ;
#50313=DIRECTION ( 'NONE',  ( -0.000000000000000000, 1.000000000000000000, -0.000000000000000000 ) ) ;
#50314=EDGE_CURVE ( 'NONE', #71164, #129204, #16414, .T. ) ;
#50315=DIRECTION ( 'NONE',  ( 0.000000000000000000, 1.000000000000000000, 0.000000000000000000 ) ) ;
#50316=DIRECTION ( 'NONE',  ( 0.000000000000000000, 0.000000000000000000, 1.000000000000000000 ) ) ;
#50317=DIRECTION ( 'NONE',  ( 0.000000000000000000, 0.000000000000000000, 1.000000000000000000 ) ) ;
#50318=DIRECTION ( 'NONE',  ( 0.000000000000000000, 0.000000000000000000, 1.000000000000000000 ) ) ;
#50319=EDGE_CURVE ( 'NONE', #58972, #49723, #43588, .T. ) ;
#50320=EDGE_CURVE ( 'NONE', #17512, #74641, #68693, .T. ) ;
#50321=ADVANCED_FACE ( 'NONE', ( #86466 ), #116712, .T. ) ;
#50322=DIRECTION ( 'NONE',  ( 0.000000000000000000, -0.9999939076577903929, 0.003490651415223739937 ) ) ;
#50323=AXIS2_PLACEMENT_3D ( 'NONE', #10539, #119864, #80595 ) ;
#50324=AXIS2_PLACEMENT_3D ( 'NONE', #50955, #10994, #90861 ) ;
#50325=ORIENTED_EDGE ( 'NONE', *, *, #91780, .T. ) ;
#50326=EDGE_CURVE ( 'NONE', #62091, #23183, #3850, .T. ) ;
#50327=ORIENTED_EDGE ( 'NONE', *, *, #87512, .F. ) ;
#50328=ORIENTED_EDGE ( 'NONE', *, *, #64738, .T. ) ;
#50329=ORIENTED_EDGE ( 'NONE', *, *, #34066, .T. ) ;
#50330=PLANE ( 'NONE',  #33692 ) ;
#50331=FACE_OUTER_BOUND ( 'NONE', #91289, .T. ) ;
#50332=CIRCLE ( 'NONE', #54518, 0.06509327318403745899 ) ;
#50334=ORIENTED_EDGE ( 'NONE', *, *, #107198, .F. ) ;
#50335=PLANE ( 'NONE',  #48607 ) ;
#50337=CARTESIAN_POINT ( 'NONE',  ( -1.700000000000034817, 12.50000000000000000, -2.385244779468109755E-15 ) ) ;
#50338=CARTESIAN_POINT ( 'NONE',  ( 7.899999999999924860, 2.500000000000000000, 5.022947341949748790 ) ) ;
#50339=ORIENTED_EDGE ( 'NONE', *, *, #14077, .F. ) ;
#50340=CARTESIAN_POINT ( 'NONE',  ( -10.45000000000000107, 2.500000000000000000, 6.595190528383296780 ) ) ;
#50341=CARTESIAN_POINT ( 'NONE',  ( -3.950000000000024603, 12.50000000000000000, -2.446380397790840266 ) ) ;
#50342=AXIS2_PLACEMENT_3D ( 'NONE', #119092, #118437, #28787 ) ;
#50343=ORIENTED_EDGE ( 'NONE', *, *, #122609, .T. ) ;
#50344=VERTEX_POINT ( 'NONE', #95653 ) ;
#50345=ORIENTED_EDGE ( 'NONE', *, *, #96751, .T. ) ;
#50346=ORIENTED_EDGE ( 'NONE', *, *, #122540, .T. ) ;
#50347=DIRECTION ( 'NONE',  ( 0.000000000000000000, 1.000000000000000000, 0.000000000000000000 ) ) ;
#50348=VECTOR ( 'NONE', #25395, 1000.000000000000000 ) ;
#50349=CARTESIAN_POINT ( 'NONE',  ( 2.499999999999948930, 2.500000000000000000, -4.922947341949753586 ) ) ;
#50350=DIRECTION ( 'NONE',  ( 0.000000000000000000, 1.000000000000000000, 0.000000000000000000 ) ) ;
#50351=AXIS2_PLACEMENT_3D ( 'NONE', #25114, #74872, #4817 ) ;
#50352=DIRECTION ( 'NONE',  ( -0.000000000000000000, 1.000000000000000000, -0.000000000000000000 ) ) ;
#50353=ORIENTED_EDGE ( 'NONE', *, *, #6157, .T. ) ;
#50354=CARTESIAN_POINT ( 'NONE',  ( -11.25000000000000178, 2.500000000000000000, -1.572243186433546214 ) ) ;
#50355=CARTESIAN_POINT ( 'NONE',  ( -5.650000000000019895, 2.500000000000000000, 6.148780366869520009 ) ) ;
#50356=DIRECTION ( 'NONE',  ( 0.000000000000000000, -0.9999939076577903929, 0.003490651415223739937 ) ) ;
#50357=CARTESIAN_POINT ( 'NONE',  ( 0.1999999999999636513, 2.500000000000000000, -0.3464101615137760715 ) ) ;
#50359=DIRECTION ( 'NONE',  ( 0.000000000000000000, -0.000000000000000000, 1.000000000000000000 ) ) ;
#50360=EDGE_CURVE ( 'NONE', #7073, #17919, #110457, .T. ) ;
#50361=ORIENTED_EDGE ( 'NONE', *, *, #51225, .F. ) ;
#50362=ORIENTED_EDGE ( 'NONE', *, *, #44709, .T. ) ;
#50363=DIRECTION ( 'NONE',  ( 0.000000000000000000, 0.000000000000000000, 1.000000000000000000 ) ) ;
#50364=DIRECTION ( 'NONE',  ( 0.000000000000000000, 0.000000000000000000, 1.000000000000000000 ) ) ;
#50365=FACE_BOUND ( 'NONE', #102275, .T. ) ;
#50366=LINE ( 'NONE', #121041, #114045 ) ;
#50367=DIRECTION ( 'NONE',  ( 0.000000000000000000, 0.000000000000000000, 1.000000000000000000 ) ) ;
#50368=CARTESIAN_POINT ( 'NONE',  ( -14.54999999999998472, 12.50000000000000000, 2.230156782645138946 ) ) ;
#50369=ADVANCED_FACE ( 'NONE', ( #85185 ), #14302, .T. ) ;
#50370=AXIS2_PLACEMENT_3D ( 'NONE', #55291, #95220, #85390 ) ;
#50371=AXIS2_PLACEMENT_3D ( 'NONE', #36159, #125795, #64949 ) ;
#50372=PLANE ( 'NONE',  #37947 ) ;
#50373=AXIS2_PLACEMENT_3D ( 'NONE', #67831, #20035, #99887 ) ;
#50374=LINE ( 'NONE', #58911, #101220 ) ;
#50375=CARTESIAN_POINT ( 'NONE',  ( -1.900000000000035438, 2.500000000000000000, 3.983716857408420076 ) ) ;
#50376=LINE ( 'NONE', #90277, #38565 ) ;
#50377=ORIENTED_EDGE ( 'NONE', *, *, #13107, .F. ) ;
#50378=DIRECTION ( 'NONE',  ( 0.000000000000000000, 0.000000000000000000, 1.000000000000000000 ) ) ;
#50379=CIRCLE ( 'NONE', #14748, 0.1000000000000002554 ) ;
#50380=DIRECTION ( 'NONE',  ( -0.000000000000000000, -1.000000000000000000, -0.000000000000000000 ) ) ;
#50381=EDGE_LOOP ( 'NONE', ( #27324, #70745 ) ) ;
#50382=EDGE_LOOP ( 'NONE', ( #67833, #115546, #115079, #72814 ) ) ;
#50383=AXIS2_PLACEMENT_3D ( 'NONE', #128039, #107752, #90026 ) ;
#50384=FACE_OUTER_BOUND ( 'NONE', #111481, .T. ) ;
#50385=FACE_OUTER_BOUND ( 'NONE', #43809, .T. ) ;
#50386=FACE_BOUND ( 'NONE', #21624, .T. ) ;
#50387=DIRECTION ( 'NONE',  ( 0.000000000000000000, 0.000000000000000000, 1.000000000000000000 ) ) ;
#50388=PLANE ( 'NONE',  #82099 ) ;
#50389=VERTEX_POINT ( 'NONE', #56999 ) ;
#50390=DIRECTION ( 'NONE',  ( 0.000000000000000000, -0.000000000000000000, 1.000000000000000000 ) ) ;
#50391=CARTESIAN_POINT ( 'NONE',  ( -3.950000000000026379, 2.500000000000000000, 2.411473670974873862 ) ) ;
#50392=EDGE_LOOP ( 'NONE', ( #72720, #49249, #52484, #112925 ) ) ;
#50393=CARTESIAN_POINT ( 'NONE',  ( -4.550000000000022915, 2.500000000000000000, -2.265063509461101798 ) ) ;
#50395=EDGE_CURVE ( 'NONE', #3248, #44501, #70756, .T. ) ;
#50396=VECTOR ( 'NONE', #107253, 1000.000000000000000 ) ;
#50397=DIRECTION ( 'NONE',  ( 0.000000000000000000, 1.000000000000000000, 0.000000000000000000 ) ) ;
#50398=DIRECTION ( 'NONE',  ( -0.000000000000000000, -1.000000000000000000, -0.000000000000000000 ) ) ;
#50399=AXIS2_PLACEMENT_3D ( 'NONE', #38597, #17631, #119071 ) ;
#50400=EDGE_CURVE ( 'NONE', #108643, #70884, #104204, .T. ) ;
#50401=AXIS2_PLACEMENT_3D ( 'NONE', #47573, #57385, #87469 ) ;
#50402=VERTEX_POINT ( 'NONE', #76007 ) ;
#50403=CARTESIAN_POINT ( 'NONE',  ( 2.499999999999948930, 12.50000000000000000, -5.088040615133791356 ) ) ;
#50404=DIRECTION ( 'NONE',  ( 0.000000000000000000, 0.000000000000000000, 1.000000000000000000 ) ) ;
#50405=DIRECTION ( 'NONE',  ( 0.000000000000000000, -0.9999939076577903929, 0.003490651415223739937 ) ) ;
#50406=CARTESIAN_POINT ( 'NONE',  ( 9.149999999999920419, 12.50000000000000000, 1.472243186433545459 ) ) ;
#50407=ORIENTED_EDGE ( 'NONE', *, *, #11743, .F. ) ;
#50408=ADVANCED_FACE ( 'NONE', ( #26277 ), #82810, .T. ) ;
#50409=ORIENTED_EDGE ( 'NONE', *, *, #123284, .F. ) ;
#50410=EDGE_CURVE ( 'NONE', #92182, #53057, #20659, .T. ) ;
#50412=AXIS2_PLACEMENT_3D ( 'NONE', #115870, #107337, #125044 ) ;
#50413=ORIENTED_EDGE ( 'NONE', *, *, #127912, .F. ) ;
#50414=DIRECTION ( 'NONE',  ( 0.000000000000000000, 0.000000000000000000, 1.000000000000000000 ) ) ;
#50415=AXIS2_PLACEMENT_3D ( 'NONE', #1997, #62233, #13743 ) ;
#50417=CARTESIAN_POINT ( 'NONE',  ( -1.900000000000034994, 2.500000000000000000, -4.776537180435978414 ) ) ;
#50418=EDGE_LOOP ( 'NONE', ( #86406, #23524, #61476, #124981 ) ) ;
#50419=ADVANCED_FACE ( 'NONE', ( #10796 ), #64578, .T. ) ;
#50420=LINE ( 'NONE', #70069, #53739 ) ;
#50421=CARTESIAN_POINT ( 'NONE',  ( -3.950000000000026379, 2.500000000000000000, -1.818653347947326138 ) ) ;
#50422=CARTESIAN_POINT ( 'NONE',  ( -5.400000000000023448, 2.500000000000000000, -4.430127018922202176 ) ) ;
#50423=DIRECTION ( 'NONE',  ( 0.000000000000000000, -0.000000000000000000, 1.000000000000000000 ) ) ;
#50424=DIRECTION ( 'NONE',  ( -0.000000000000000000, 1.000000000000000000, -0.000000000000000000 ) ) ;
#50425=EDGE_CURVE ( 'NONE', #98142, #4651, #22607, .T. ) ;
#50426=DIRECTION ( 'NONE',  ( 0.000000000000000000, 0.000000000000000000, 1.000000000000000000 ) ) ;
#50427=AXIS2_PLACEMENT_3D ( 'NONE', #104595, #24114, #103967 ) ;
#50428=ORIENTED_EDGE ( 'NONE', *, *, #9847, .T. ) ;
#50429=AXIS2_PLACEMENT_3D ( 'NONE', #102385, #69691, #50081 ) ;
#50430=ORIENTED_EDGE ( 'NONE', *, *, #7725, .T. ) ;
#50431=CARTESIAN_POINT ( 'NONE',  ( -0.4000000000000392131, 2.500000000000000000, -4.230127018922201998 ) ) ;
#50432=EDGE_LOOP ( 'NONE', ( #85853, #2608 ) ) ;
#50434=EDGE_LOOP ( 'NONE', ( #42663, #76054, #76754, #46943 ) ) ;
#50435=ORIENTED_EDGE ( 'NONE', *, *, #56897, .T. ) ;
#50436=ORIENTED_EDGE ( 'NONE', *, *, #19385, .T. ) ;
#50437=DIRECTION ( 'NONE',  ( -0.000000000000000000, -1.000000000000000000, -0.000000000000000000 ) ) ;
#50438=DIRECTION ( 'NONE',  ( 0.000000000000000000, 0.000000000000000000, 1.000000000000000000 ) ) ;
#50439=DIRECTION ( 'NONE',  ( 0.000000000000000000, 1.000000000000000000, 0.000000000000000000 ) ) ;
#50441=CARTESIAN_POINT ( 'NONE',  ( 2.899999999999945732, 12.50000000000000000, -2.385244779468109755E-15 ) ) ;
#50442=VECTOR ( 'NONE', #12073, 1000.000000000000000 ) ;
#50443=AXIS2_PLACEMENT_3D ( 'NONE', #113073, #33869, #94087 ) ;
#50444=CARTESIAN_POINT ( 'NONE',  ( 11.89999999999990798, 12.50000000000000000, -4.741630453620015118 ) ) ;
#50445=DIRECTION ( 'NONE',  ( 0.000000000000000000, 1.000000000000000000, 0.000000000000000000 ) ) ;
#50446=CARTESIAN_POINT ( 'NONE',  ( 2.499999999999981792, 2.500000000000000000, 4.330127018922196314 ) ) ;
#50447=CARTESIAN_POINT ( 'NONE',  ( 8.749999999999953815, 2.500000000000000000, -2.065063509461102065 ) ) ;
#50448=FACE_OUTER_BOUND ( 'NONE', #102589, .T. ) ;
#50449=EDGE_LOOP ( 'NONE', ( #59432, #98999 ) ) ;
#50450=EDGE_CURVE ( 'NONE', #42165, #86633, #68789, .T. ) ;
#50451=DIRECTION ( 'NONE',  ( 0.000000000000000000, -0.000000000000000000, 1.000000000000000000 ) ) ;
#50452=ORIENTED_EDGE ( 'NONE', *, *, #82224, .F. ) ;
#50453=ORIENTED_EDGE ( 'NONE', *, *, #12458, .F. ) ;
#50454=LINE ( 'NONE', #29537, #31504 ) ;
#50455=FACE_OUTER_BOUND ( 'NONE', #24795, .T. ) ;
#50456=EDGE_CURVE ( 'NONE', #47635, #31556, #31159, .T. ) ;
#50458=FACE_OUTER_BOUND ( 'NONE', #123283, .T. ) ;
#50459=DIRECTION ( 'NONE',  ( -4.274815082592931898E-19, -0.9999939076577903929, -0.003490651415223739937 ) ) ;
#50460=AXIS2_PLACEMENT_3D ( 'NONE', #122433, #111290, #72047 ) ;
#50461=CARTESIAN_POINT ( 'NONE',  ( -4.550000000000026468, 2.500000000000000000, -6.495190528383302464 ) ) ;
#50462=ORIENTED_EDGE ( 'NONE', *, *, #16740, .T. ) ;
#50463=CONICAL_SURFACE ( 'NONE', #60930, 0.1000000000000000472, 0.003490658503988666988 ) ;
#50464=EDGE_CURVE ( 'NONE', #4878, #85926, #33304, .T. ) ;
#50465=CONICAL_SURFACE ( 'NONE', #87999, 0.1000000000000002554, 0.003490658503988666988 ) ;
#50466=EDGE_CURVE ( 'NONE', #74459, #13178, #2951, .T. ) ;
#50467=ADVANCED_FACE ( 'NONE', ( #70397 ), #52688, .T. ) ;
#50468=VERTEX_POINT ( 'NONE', #51423 ) ;
#50469=CARTESIAN_POINT ( 'NONE',  ( -5.650000000000019895, 2.500000000000000000, 6.741600689897071952 ) ) ;
#50470=CONICAL_SURFACE ( 'NONE', #81762, 0.1000000000000002554, 0.003490658503988666988 ) ;
#50471=ORIENTED_EDGE ( 'NONE', *, *, #29993, .F. ) ;
#50472=CIRCLE ( 'NONE', #85955, 0.1000000000000000056 ) ;
#50473=DIRECTION ( 'NONE',  ( 0.000000000000000000, 0.000000000000000000, 1.000000000000000000 ) ) ;
#50474=EDGE_CURVE ( 'NONE', #73263, #34057, #26938, .T. ) ;
#50475=ORIENTED_EDGE ( 'NONE', *, *, #4781, .T. ) ;
#50476=AXIS2_PLACEMENT_3D ( 'NONE', #19196, #38227, #78805 ) ;
#50477=ORIENTED_EDGE ( 'NONE', *, *, #114551, .F. ) ;
#50478=CARTESIAN_POINT ( 'NONE',  ( 2.499999999999947153, 12.50000000000000000, 3.572213422710607489 ) ) ;
#50479=DIRECTION ( 'NONE',  ( -0.000000000000000000, 1.000000000000000000, -0.000000000000000000 ) ) ;
#50481=ADVANCED_FACE ( 'NONE', ( #41602 ), #75054, .T. ) ;
#50482=DIRECTION ( 'NONE',  ( 0.000000000000000000, -0.9999939076577903929, 0.003490651415223739937 ) ) ;
#50483=PLANE ( 'NONE',  #77910 ) ;
#50484=CARTESIAN_POINT ( 'NONE',  ( 17.50000000000000000, 1.666666666666665186, 4.000000000000000000 ) ) ;
#50485=VERTEX_POINT ( 'NONE', #42236 ) ;
#50486=DIRECTION ( 'NONE',  ( 0.000000000000000000, 1.000000000000000000, 0.000000000000000000 ) ) ;
#50487=CARTESIAN_POINT ( 'NONE',  ( 0.7999999999999548583, 2.500000000000000000, 4.230127018922196669 ) ) ;
#50488=CARTESIAN_POINT ( 'NONE',  ( 8.349999999999919709, 2.500000000000000000, -2.857883832488653741 ) ) ;
#50489=DIRECTION ( 'NONE',  ( 0.000000000000000000, 1.000000000000000000, 0.000000000000000000 ) ) ;
#50490=DIRECTION ( 'NONE',  ( 0.000000000000000000, 0.000000000000000000, 1.000000000000000000 ) ) ;
#50491=ORIENTED_EDGE ( 'NONE', *, *, #22569, .F. ) ;
#50492=ORIENTED_EDGE ( 'NONE', *, *, #1803, .T. ) ;
#50493=CARTESIAN_POINT ( 'NONE',  ( -3.750000000000025757, 12.50000000000000000, -2.857883832488653741 ) ) ;
#50494=EDGE_LOOP ( 'NONE', ( #89489, #111546 ) ) ;
#50495=CARTESIAN_POINT ( 'NONE',  ( 14.39999999999989555, 2.500000000000000000, 0.4464101615137736623 ) ) ;
#50496=DIRECTION ( 'NONE',  ( 0.000000000000000000, 1.000000000000000000, 0.000000000000000000 ) ) ;
#50497=AXIS2_PLACEMENT_3D ( 'NONE', #93781, #63684, #91200 ) ;
#50499=CARTESIAN_POINT ( 'NONE',  ( 3.749999999999944045, 12.50000000000000000, -2.857883832488653741 ) ) ;
#50500=CARTESIAN_POINT ( 'NONE',  ( -8.350000000000008527, 2.500000000000000000, 7.188010851410848723 ) ) ;
#50501=CARTESIAN_POINT ( 'NONE',  ( 11.04999999999990656, 12.50000000000000000, 2.511473670974873507 ) ) ;
#50502=CARTESIAN_POINT ( 'NONE',  ( -5.850000000000018296, 12.50000000000000000, 1.472243186433545459 ) ) ;
#50503=CONICAL_SURFACE ( 'NONE', #60970, 0.1000000000000000056, 0.003490658503988666988 ) ;
#50504=AXIS2_PLACEMENT_3D ( 'NONE', #18268, #79771, #29398 ) ;
#50505=CARTESIAN_POINT ( 'NONE',  ( 9.799999999999917222, 2.500000000000000000, 0.2464101615137735679 ) ) ;
#50506=AXIS2_PLACEMENT_3D ( 'NONE', #118907, #16809, #67191 ) ;
#50507=ORIENTED_EDGE ( 'NONE', *, *, #66981, .T. ) ;
#50508=CARTESIAN_POINT ( 'NONE',  ( 59.88498294812150391, 2.860410289928506433, -5.641291750192007903 ) ) ;
#50509=CARTESIAN_POINT ( 'NONE',  ( 4.349999999999938360, 2.500000000000000000, 1.918653347947321564 ) ) ;
#50510=CARTESIAN_POINT ( 'NONE',  ( -9.999999999999969802, 12.50000000000000000, 4.395220292106234439 ) ) ;
#50511=AXIS2_PLACEMENT_3D ( 'NONE', #118632, #27043, #87869 ) ;
#50512=DIRECTION ( 'NONE',  ( 0.000000000000000000, 0.000000000000000000, 1.000000000000000000 ) ) ;
#50513=EDGE_CURVE ( 'NONE', #113633, #44909, #114747, .T. ) ;
#50514=ORIENTED_EDGE ( 'NONE', *, *, #32506, .T. ) ;
#50515=CIRCLE ( 'NONE', #67209, 0.06509327318403745899 ) ;
#50516=EDGE_LOOP ( 'NONE', ( #53355, #41446, #101556, #92113 ) ) ;
#50517=LINE ( 'NONE', #82581, #16599 ) ;
#50518=DIRECTION ( 'NONE',  ( 0.000000000000000000, 0.000000000000000000, -1.000000000000000000 ) ) ;
#50519=CIRCLE ( 'NONE', #52584, 0.09999999999999982514 ) ;
#50520=FACE_OUTER_BOUND ( 'NONE', #60706, .T. ) ;
#50521=ORIENTED_EDGE ( 'NONE', *, *, #71456, .T. ) ;
#50522=CARTESIAN_POINT ( 'NONE',  ( -8.550000000000013145, 12.50000000000000000, -1.753560074763288679 ) ) ;
#50523=CARTESIAN_POINT ( 'NONE',  ( -3.749999999999991118, 2.500000000000000000, -2.265063509461101798 ) ) ;
#50524=AXIS2_PLACEMENT_3D ( 'NONE', #59099, #30300, #78755 ) ;
#50525=CIRCLE ( 'NONE', #35871, 0.1000000000000002554 ) ;
#50526=ORIENTED_EDGE ( 'NONE', *, *, #107770, .F. ) ;
#50527=CARTESIAN_POINT ( 'NONE',  ( 6.649999999999931077, 12.50000000000000000, -6.495190528383302464 ) ) ;
#50528=ORIENTED_EDGE ( 'NONE', *, *, #108262, .F. ) ;
#50529=CARTESIAN_POINT ( 'NONE',  ( -8.550000000000013145, 2.500000000000000000, 2.411473670974873862 ) ) ;
#50530=VERTEX_POINT ( 'NONE', #72347 ) ;
#50531=CARTESIAN_POINT ( 'NONE',  ( 8.349999999999919709, 12.50000000000000000, 6.495190528383297135 ) ) ;
#50532=CARTESIAN_POINT ( 'NONE',  ( 4.848431875627500887, 2.499999999999999112, -8.943854603337394238 ) ) ;
#50533=ORIENTED_EDGE ( 'NONE', *, *, #41160, .F. ) ;
#50535=DIRECTION ( 'NONE',  ( 0.000000000000000000, 1.000000000000000000, 0.000000000000000000 ) ) ;
#50536=CARTESIAN_POINT ( 'NONE',  ( -0.6000000000000383915, 12.50000000000000000, -4.048810130592463530 ) ) ;
#50537=EDGE_LOOP ( 'NONE', ( #66290, #96303 ) ) ;
#50538=DIRECTION ( 'NONE',  ( 0.000000000000000000, 0.000000000000000000, 1.000000000000000000 ) ) ;
#50539=DIRECTION ( 'NONE',  ( -4.274815082592931898E-19, -0.9999939076577903929, -0.003490651415223739937 ) ) ;
#50540=FACE_OUTER_BOUND ( 'NONE', #91578, .T. ) ;
#50541=AXIS2_PLACEMENT_3D ( 'NONE', #42510, #129607, #62146 ) ;
#50543=DIRECTION ( 'NONE',  ( -0.000000000000000000, -1.000000000000000000, -0.000000000000000000 ) ) ;
#50544=AXIS2_PLACEMENT_3D ( 'NONE', #83318, #3456, #45327 ) ;
#50545=DIRECTION ( 'NONE',  ( 0.000000000000000000, -0.000000000000000000, 1.000000000000000000 ) ) ;
#50546=CARTESIAN_POINT ( 'NONE',  ( -9.600000000000008527, 2.500000000000000000, 4.330127018922196314 ) ) ;
#50547=EDGE_CURVE ( 'NONE', #117651, #51156, #99865, .T. ) ;
#50548=CONICAL_SURFACE ( 'NONE', #69327, 0.1000000000000002554, 0.003490658503988666988 ) ;
#50549=EDGE_LOOP ( 'NONE', ( #93270, #90848 ) ) ;
#50550=AXIS2_PLACEMENT_3D ( 'NONE', #20021, #12743, #120147 ) ;
#50551=ORIENTED_EDGE ( 'NONE', *, *, #88125, .T. ) ;
#50552=EDGE_LOOP ( 'NONE', ( #99460, #8536, #9, #97259 ) ) ;
#50553=LINE ( 'NONE', #71486, #106047 ) ;
#50554=DIRECTION ( 'NONE',  ( 0.000000000000000000, 0.000000000000000000, -1.000000000000000000 ) ) ;
#50556=CARTESIAN_POINT ( 'NONE',  ( -11.69999999999999929, 2.500000000000000000, -4.330127018922198978 ) ) ;
#50557=AXIS2_PLACEMENT_3D ( 'NONE', #17823, #26375, #65638 ) ;
#50558=ORIENTED_EDGE ( 'NONE', *, *, #13938, .F. ) ;
#50559=ORIENTED_EDGE ( 'NONE', *, *, #14551, .T. ) ;
#50560=EDGE_CURVE ( 'NONE', #12189, #68896, #29102, .T. ) ;
#50561=FACE_BOUND ( 'NONE', #95853, .T. ) ;
#50562=ORIENTED_EDGE ( 'NONE', *, *, #98320, .F. ) ;
#50563=EDGE_CURVE ( 'NONE', #10632, #26142, #120780, .T. ) ;
#50564=CARTESIAN_POINT ( 'NONE',  ( 6.849999999999929479, 2.500000000000000000, 6.841600689897072485 ) ) ;
#50565=DIRECTION ( 'NONE',  ( 0.000000000000000000, 0.000000000000000000, -1.000000000000000000 ) ) ;
#50566=AXIS2_PLACEMENT_3D ( 'NONE', #127362, #28515, #39007 ) ;
#50567=DIRECTION ( 'NONE',  ( 0.000000000000000000, 0.000000000000000000, 1.000000000000000000 ) ) ;
#50568=DIRECTION ( 'NONE',  ( -0.000000000000000000, 1.000000000000000000, -0.000000000000000000 ) ) ;
#50569=CARTESIAN_POINT ( 'NONE',  ( -3.350000000000028955, 12.50000000000000000, 7.188010851410848723 ) ) ;
#50570=CARTESIAN_POINT ( 'NONE',  ( 13.94999999999989804, 12.50000000000000000, 1.818653347947321475 ) ) ;
#50571=ADVANCED_FACE ( 'NONE', ( #21287 ), #6074, .T. ) ;
#50572=DIRECTION ( 'NONE',  ( 0.000000000000000000, 1.000000000000000000, 0.000000000000000000 ) ) ;
#50573=EDGE_CURVE ( 'NONE', #39206, #28200, #125226, .T. ) ;
#50574=CARTESIAN_POINT ( 'NONE',  ( -3.350000000000028511, 2.500000000000000000, 1.572243186433545548 ) ) ;
#50575=ADVANCED_FACE ( 'NONE', ( #94537 ), #110551, .T. ) ;
#50576=CARTESIAN_POINT ( 'NONE',  ( -6.250000000000019540, 12.50000000000000000, -2.857883832488653741 ) ) ;
#50577=EDGE_CURVE ( 'NONE', #120557, #112512, #72996, .T. ) ;
#50578=CARTESIAN_POINT ( 'NONE',  ( 10.19999999999991225, 12.50000000000000000, 3.983716857408420076 ) ) ;
#50579=EDGE_LOOP ( 'NONE', ( #115909, #103982, #21186, #112766 ) ) ;
#50580=VERTEX_POINT ( 'NONE', #54601 ) ;
#50581=VERTEX_POINT ( 'NONE', #85989 ) ;
#50583=DIRECTION ( 'NONE',  ( 0.000000000000000000, -0.9999939076577903929, 0.003490651415223739937 ) ) ;
#50584=FACE_OUTER_BOUND ( 'NONE', #78125, .T. ) ;
#50585=ORIENTED_EDGE ( 'NONE', *, *, #11565, .F. ) ;
#50586=VERTEX_POINT ( 'NONE', #33071 ) ;
#50587=VERTEX_POINT ( 'NONE', #95839 ) ;
#50588=CARTESIAN_POINT ( 'NONE',  ( -6.050000000000020250, 2.500000000000000000, -2.411473670974877859 ) ) ;
#50589=VECTOR ( 'NONE', #51931, 1000.000000000000000 ) ;
#50590=CARTESIAN_POINT ( 'NONE',  ( 3.099999999999944134, 2.500000000000000000, 4.676537180435972552 ) ) ;
#50591=DIRECTION ( 'NONE',  ( 0.000000000000000000, 0.000000000000000000, -1.000000000000000000 ) ) ;
#50592=CARTESIAN_POINT ( 'NONE',  ( 13.74999999999989697, 12.50000000000000000, 2.857883832488649301 ) ) ;
#50593=DIRECTION ( 'NONE',  ( 0.000000000000000000, 0.000000000000000000, 1.000000000000000000 ) ) ;
#50594=CARTESIAN_POINT ( 'NONE',  ( 5.649999999999934630, 2.500000000000000000, -1.818653347947325916 ) ) ;
#50595=DIRECTION ( 'NONE',  ( -4.274815082592931898E-19, -0.9999939076577903929, -0.003490651415223739937 ) ) ;
#50596=VERTEX_POINT ( 'NONE', #74912 ) ;
#50597=CIRCLE ( 'NONE', #125798, 0.09999999999999982514 ) ;
#50598=CIRCLE ( 'NONE', #58925, 0.1000000000000002554 ) ;
#50599=CARTESIAN_POINT ( 'NONE',  ( 13.34999999999989662, 2.500000000000000000, -2.757883832488654097 ) ) ;
#50600=ORIENTED_EDGE ( 'NONE', *, *, #41208, .T. ) ;
#50601=VECTOR ( 'NONE', #20383, 1000.000000000000000 ) ;
#50602=ORIENTED_EDGE ( 'NONE', *, *, #81991, .F. ) ;
#50603=CIRCLE ( 'NONE', #71533, 0.09999999999999982514 ) ;
#50604=ORIENTED_EDGE ( 'NONE', *, *, #65044, .T. ) ;
#50605=DIRECTION ( 'NONE',  ( 0.000000000000000000, -0.9999939076577903929, 0.003490651415223739937 ) ) ;
#50606=EDGE_CURVE ( 'NONE', #38108, #68087, #4859, .T. ) ;
#50607=ORIENTED_EDGE ( 'NONE', *, *, #96693, .T. ) ;
#50608=ORIENTED_EDGE ( 'NONE', *, *, #10873, .F. ) ;
#50609=FACE_OUTER_BOUND ( 'NONE', #83901, .T. ) ;
#50610=AXIS2_PLACEMENT_3D ( 'NONE', #32218, #2073, #69530 ) ;
#50611=LINE ( 'NONE', #80739, #127033 ) ;
#50612=CARTESIAN_POINT ( 'NONE',  ( 3.749999999999942268, 2.500000000000000000, -1.572243186433550211 ) ) ;
#50613=DIRECTION ( 'NONE',  ( 0.000000000000000000, 1.000000000000000000, 0.000000000000000000 ) ) ;
#50614=CIRCLE ( 'NONE', #92370, 0.09999999999999999167 ) ;
#50615=DIRECTION ( 'NONE',  ( -0.000000000000000000, 1.000000000000000000, -0.000000000000000000 ) ) ;
#50616=CIRCLE ( 'NONE', #52675, 0.06509327318403745899 ) ;
#50617=AXIS2_PLACEMENT_3D ( 'NONE', #26289, #5339, #85195 ) ;
#50618=EDGE_CURVE ( 'NONE', #52298, #89250, #4212, .T. ) ;
#50619=CARTESIAN_POINT ( 'NONE',  ( 10.39999999999991154, 2.500000000000000000, -5.122947341949753763 ) ) ;
#50620=EDGE_CURVE ( 'NONE', #98964, #129208, #77110, .T. ) ;
#50621=CONICAL_SURFACE ( 'NONE', #75747, 0.1000000000000002554, 0.003490658503988666988 ) ;
#50622=EDGE_CURVE ( 'NONE', #69752, #18522, #23215, .T. ) ;
#50623=CARTESIAN_POINT ( 'NONE',  ( -11.64999999999999680, 2.500000000000000000, -6.595190528383298556 ) ) ;
#50624=EDGE_LOOP ( 'NONE', ( #4245, #83910, #91210, #28473 ) ) ;
#50625=CARTESIAN_POINT ( 'NONE',  ( 21.24748442509683244, -0.7426088330904641044, 4.181982359507943947 ) ) ;
#50626=EDGE_CURVE ( 'NONE', #122009, #78632, #1882, .T. ) ;
#50627=ORIENTED_EDGE ( 'NONE', *, *, #44074, .F. ) ;
#50630=CARTESIAN_POINT ( 'NONE',  ( -9.800000000000004263, 2.500000000000000000, 4.083716857408420609 ) ) ;
#50631=ADVANCED_FACE ( 'NONE', ( #55903 ), #49941, .T. ) ;
#50632=ORIENTED_EDGE ( 'NONE', *, *, #95252, .F. ) ;
#50633=DIRECTION ( 'NONE',  ( 0.000000000000000000, 0.000000000000000000, 1.000000000000000000 ) ) ;
#50634=EDGE_CURVE ( 'NONE', #8778, #58319, #123174, .T. ) ;
#50636=ORIENTED_EDGE ( 'NONE', *, *, #58041, .F. ) ;
#50637=EDGE_CURVE ( 'NONE', #33308, #118779, #47878, .T. ) ;
#50638=EDGE_CURVE ( 'NONE', #99278, #84066, #3941, .T. ) ;
#50639=EDGE_CURVE ( 'NONE', #89885, #90718, #118960, .T. ) ;
#50640=CARTESIAN_POINT ( 'NONE',  ( -0.8500000000000382805, 2.500000000000000000, -1.472243186433550122 ) ) ;
#50641=ORIENTED_EDGE ( 'NONE', *, *, #9115, .T. ) ;
#50642=ORIENTED_EDGE ( 'NONE', *, *, #91346, .F. ) ;
#50643=DIRECTION ( 'NONE',  ( -0.000000000000000000, -1.000000000000000000, -0.000000000000000000 ) ) ;
#50644=CARTESIAN_POINT ( 'NONE',  ( 11.44999999999990514, 12.50000000000000000, -6.148780366869526226 ) ) ;
#50645=CARTESIAN_POINT ( 'NONE',  ( 9.349999999999919709, 2.500000000000000000, -6.048780366869526581 ) ) ;
#50646=LINE ( 'NONE', #61110, #93154 ) ;
#50647=EDGE_CURVE ( 'NONE', #52447, #6702, #37413, .T. ) ;
#50648=LINE ( 'NONE', #101040, #56204 ) ;
#50649=EDGE_LOOP ( 'NONE', ( #76413, #75055, #45119, #55080 ) ) ;
#50650=DIRECTION ( 'NONE',  ( 0.000000000000000000, -0.9999939076577903929, 0.003490651415223739937 ) ) ;
#50651=CIRCLE ( 'NONE', #98658, 0.09999999999999999167 ) ;
#50652=AXIS2_PLACEMENT_3D ( 'NONE', #107507, #95756, #17828 ) ;
#50653=AXIS2_PLACEMENT_3D ( 'NONE', #16473, #28906, #77352 ) ;
#50654=EDGE_LOOP ( 'NONE', ( #87787, #77938, #84222, #121808 ) ) ;
#50655=LINE ( 'NONE', #109588, #25653 ) ;
#50656=CARTESIAN_POINT ( 'NONE',  ( -8.100000000000013856, 2.500000000000000000, -0.2464101615137782308 ) ) ;
#50657=AXIS2_PLACEMENT_3D ( 'NONE', #24772, #64682, #126184 ) ;
#50658=CIRCLE ( 'NONE', #71480, 0.06509327318403745899 ) ;
#50659=AXIS2_PLACEMENT_3D ( 'NONE', #77964, #68138, #98892 ) ;
#50660=AXIS2_PLACEMENT_3D ( 'NONE', #24513, #75525, #84716 ) ;
#50661=CONICAL_SURFACE ( 'NONE', #96611, 0.1000000000000002554, 0.003490658503988666988 ) ;
#50663=DIRECTION ( 'NONE',  ( 0.000000000000000000, 0.000000000000000000, -1.000000000000000000 ) ) ;
#50664=FACE_OUTER_BOUND ( 'NONE', #82553, .T. ) ;
#50665=DIRECTION ( 'NONE',  ( -0.000000000000000000, -1.000000000000000000, -0.000000000000000000 ) ) ;
#50666=CARTESIAN_POINT ( 'NONE',  ( 6.849999999999930367, 2.500000000000000000, -6.841600689897078702 ) ) ;
#50668=DIRECTION ( 'NONE',  ( -0.000000000000000000, 1.000000000000000000, -0.000000000000000000 ) ) ;
#50669=CARTESIAN_POINT ( 'NONE',  ( 6.699999999999930012, 12.50000000000000000, -4.265033745738164406 ) ) ;
#50670=DIRECTION ( 'NONE',  ( 0.000000000000000000, 0.000000000000000000, -1.000000000000000000 ) ) ;
#50671=ORIENTED_EDGE ( 'NONE', *, *, #76302, .T. ) ;
#50672=DIRECTION ( 'NONE',  ( 0.000000000000000000, 0.000000000000000000, -1.000000000000000000 ) ) ;
#50673=AXIS2_PLACEMENT_3D ( 'NONE', #105073, #72419, #5578 ) ;
#50675=ORIENTED_EDGE ( 'NONE', *, *, #91149, .F. ) ;
#50676=EDGE_LOOP ( 'NONE', ( #37301, #65209, #9219, #85370 ) ) ;
#50677=CARTESIAN_POINT ( 'NONE',  ( 3.349999999999942801, 2.500000000000000000, 2.757883832488649656 ) ) ;
#50678=ORIENTED_EDGE ( 'NONE', *, *, #36751, .T. ) ;
#50679=DIRECTION ( 'NONE',  ( 0.000000000000000000, 1.000000000000000000, 0.000000000000000000 ) ) ;
#50680=DIRECTION ( 'NONE',  ( 0.000000000000000000, 0.000000000000000000, -1.000000000000000000 ) ) ;
#50681=VECTOR ( 'NONE', #78203, 1000.000000000000000 ) ;
#50682=ORIENTED_EDGE ( 'NONE', *, *, #1976, .F. ) ;
#50683=CONICAL_SURFACE ( 'NONE', #25846, 0.1000000000000002554, 0.003490658503988666988 ) ;
#50684=CARTESIAN_POINT ( 'NONE',  ( -6.250000000000021316, 2.500000000000000000, -1.472243186433550122 ) ) ;
#50685=DIRECTION ( 'NONE',  ( -0.000000000000000000, 1.000000000000000000, -0.000000000000000000 ) ) ;
#50686=LINE ( 'NONE', #36706, #107215 ) ;
#50687=EDGE_CURVE ( 'NONE', #82670, #85004, #83375, .T. ) ;
#50688=VECTOR ( 'NONE', #33777, 1000.000000000000000 ) ;
#50689=VERTEX_POINT ( 'NONE', #5501 ) ;
#50690=AXIS2_PLACEMENT_3D ( 'NONE', #40163, #11340, #80736 ) ;
#50691=AXIS2_PLACEMENT_3D ( 'NONE', #33533, #83894, #114644 ) ;
#50692=VECTOR ( 'NONE', #125979, 1000.000000000000000 ) ;
#50693=ORIENTED_EDGE ( 'NONE', *, *, #75452, .T. ) ;
#50694=ORIENTED_EDGE ( 'NONE', *, *, #95561, .T. ) ;
#50695=DIRECTION ( 'NONE',  ( 0.000000000000000000, 0.000000000000000000, 1.000000000000000000 ) ) ;
#50696=DIRECTION ( 'NONE',  ( 0.000000000000000000, 0.000000000000000000, -1.000000000000000000 ) ) ;
#50697=CARTESIAN_POINT ( 'NONE',  ( -10.20000000000000284, 2.500000000000000000, 3.883716857408421319 ) ) ;
#50698=FACE_BOUND ( 'NONE', #111592, .T. ) ;
#50699=ORIENTED_EDGE ( 'NONE', *, *, #17137, .F. ) ;
#50700=FACE_OUTER_BOUND ( 'NONE', #4865, .T. ) ;
#50701=CARTESIAN_POINT ( 'NONE',  ( 15.59999999999988951, 2.500000000000000000, 0.2464101615137735679 ) ) ;
#50702=AXIS2_PLACEMENT_3D ( 'NONE', #121042, #22223, #103350 ) ;
#50703=EDGE_LOOP ( 'NONE', ( #27466, #84094 ) ) ;
#50704=CONICAL_SURFACE ( 'NONE', #517, 0.1000000000000002554, 0.003490658503988666988 ) ;
#50705=CARTESIAN_POINT ( 'NONE',  ( -12.89999999999999325, 2.500000000000000000, -3.637306695894647390 ) ) ;
#50706=CARTESIAN_POINT ( 'NONE',  ( -10.20000000000000462, 12.50000000000000000, 4.741630453620009789 ) ) ;
#50707=AXIS2_PLACEMENT_3D ( 'NONE', #7129, #74600, #66701 ) ;
#50708=AXIS2_PLACEMENT_3D ( 'NONE', #33415, #124996, #83155 ) ;
#50709=VECTOR ( 'NONE', #61551, 1000.000000000000000 ) ;
#50710=CARTESIAN_POINT ( 'NONE',  ( -0.4000000000000404898, 2.500000000000000000, 5.022947341949748790 ) ) ;
#50711=FACE_OUTER_BOUND ( 'NONE', #13881, .T. ) ;
#50712=DIRECTION ( 'NONE',  ( 0.000000000000000000, 0.000000000000000000, 1.000000000000000000 ) ) ;
#50713=CARTESIAN_POINT ( 'NONE',  ( -6.650000000000019007, 2.500000000000000000, -1.472243186433550122 ) ) ;
#50714=CIRCLE ( 'NONE', #96665, 0.1000000000000002554 ) ;
#50715=LINE ( 'NONE', #88707, #12680 ) ;
#50716=ADVANCED_FACE ( 'NONE', ( #74266 ), #105662, .T. ) ;
#50717=ORIENTED_EDGE ( 'NONE', *, *, #72716, .T. ) ;
#50718=AXIS2_PLACEMENT_3D ( 'NONE', #111234, #22254, #1298 ) ;
#50719=ORIENTED_EDGE ( 'NONE', *, *, #3601, .T. ) ;
#50720=ORIENTED_EDGE ( 'NONE', *, *, #8733, .T. ) ;
#50721=EDGE_LOOP ( 'NONE', ( #123987, #39472, #94502, #94841 ) ) ;
#50723=DIRECTION ( 'NONE',  ( 0.000000000000000000, 0.000000000000000000, 1.000000000000000000 ) ) ;
#50724=ORIENTED_EDGE ( 'NONE', *, *, #49406, .T. ) ;
#50725=FACE_BOUND ( 'NONE', #48301, .T. ) ;
#50726=EDGE_CURVE ( 'NONE', #72665, #12542, #75533, .T. ) ;
#50727=CARTESIAN_POINT ( 'NONE',  ( 0.3999999999999559464, 2.500000000000000000, -4.430127018922202176 ) ) ;
#50728=CARTESIAN_POINT ( 'NONE',  ( -4.400000000000028777, 2.500000000000000000, -3.883716857408426648 ) ) ;
#50729=CARTESIAN_POINT ( 'NONE',  ( -6.700000000000019718, 2.500000000000000000, -4.430127018922202176 ) ) ;
#50730=DIRECTION ( 'NONE',  ( -0.000000000000000000, -1.000000000000000000, -0.000000000000000000 ) ) ;
#50731=EDGE_CURVE ( 'NONE', #1776, #8661, #70844, .T. ) ;
#50732=DIRECTION ( 'NONE',  ( 0.000000000000000000, 0.000000000000000000, 1.000000000000000000 ) ) ;
#50733=EDGE_CURVE ( 'NONE', #118880, #104652, #75142, .T. ) ;
#50734=LINE ( 'NONE', #21266, #97737 ) ;
#50735=CARTESIAN_POINT ( 'NONE',  ( -5.600000000000020073, 12.50000000000000000, 0.4115034346978110880 ) ) ;
#50736=CONICAL_SURFACE ( 'NONE', #119982, 0.1000000000000002554, 0.003490658503988666988 ) ;
#50737=ADVANCED_FACE ( 'NONE', ( #57199 ), #100192, .T. ) ;
#50738=DIRECTION ( 'NONE',  ( -0.000000000000000000, -1.000000000000000000, -0.000000000000000000 ) ) ;
#50739=ADVANCED_FACE ( 'NONE', ( #68297 ), #99066, .T. ) ;
#50741=EDGE_CURVE ( 'NONE', #99983, #120284, #10301, .T. ) ;
#50742=EDGE_LOOP ( 'NONE', ( #17426, #60129 ) ) ;
#50743=VERTEX_POINT ( 'NONE', #117373 ) ;
#50744=VERTEX_POINT ( 'NONE', #68949 ) ;
#50745=EDGE_LOOP ( 'NONE', ( #1606, #33817 ) ) ;
#50746=CONICAL_SURFACE ( 'NONE', #121742, 0.1000000000000000472, 0.003490658503988666988 ) ;
#50747=VERTEX_POINT ( 'NONE', #97122 ) ;
#50748=VECTOR ( 'NONE', #11128, 1000.000000000000000 ) ;
#50749=CIRCLE ( 'NONE', #123891, 0.09999999999999982514 ) ;
#50750=DIRECTION ( 'NONE',  ( 0.000000000000000000, 1.000000000000000000, 0.000000000000000000 ) ) ;
#50751=VERTEX_POINT ( 'NONE', #49339 ) ;
#50752=ADVANCED_FACE ( 'NONE', ( #87923 ), #58431, .T. ) ;
#50753=EDGE_CURVE ( 'NONE', #63286, #35370, #37502, .T. ) ;
#50754=AXIS2_PLACEMENT_3D ( 'NONE', #51126, #122436, #112614 ) ;
#50755=EDGE_CURVE ( 'NONE', #110598, #18873, #27099, .T. ) ;
#50756=CIRCLE ( 'NONE', #40299, 0.09999999999999982514 ) ;
#50757=CARTESIAN_POINT ( 'NONE',  ( -2.900000000000030553, 2.500000000000000000, 5.022947341949748790 ) ) ;
#50759=DIRECTION ( 'NONE',  ( -0.000000000000000000, 1.000000000000000000, -0.000000000000000000 ) ) ;
#50760=CARTESIAN_POINT ( 'NONE',  ( 5.399999999999934630, 2.500000000000000000, 0.6928203230275494784 ) ) ;
#50761=CIRCLE ( 'NONE', #21513, 0.1000000000000002554 ) ;
#50762=CIRCLE ( 'NONE', #71685, 1.000000000000000444 ) ;
#50763=AXIS2_PLACEMENT_3D ( 'NONE', #78798, #47392, #15484 ) ;
#50764=EDGE_LOOP ( 'NONE', ( #126586, #78355, #57902, #94204 ) ) ;
#50765=CARTESIAN_POINT ( 'NONE',  ( -11.25000000000000000, 2.500000000000000000, -7.188010851410850499 ) ) ;
#50766=AXIS2_PLACEMENT_3D ( 'NONE', #82860, #10849, #91370 ) ;
#50767=EDGE_LOOP ( 'NONE', ( #111502, #52046 ) ) ;
#50768=VERTEX_POINT ( 'NONE', #67001 ) ;
#50769=CARTESIAN_POINT ( 'NONE',  ( 5.849999999999933920, 2.500000000000000000, -2.957883832488653830 ) ) ;
#50770=CARTESIAN_POINT ( 'NONE',  ( -0.6000000000000388356, 12.50000000000000000, 3.983716857408420964 ) ) ;
#50771=DIRECTION ( 'NONE',  ( 0.000000000000000000, 0.000000000000000000, 1.000000000000000000 ) ) ;
#50772=ORIENTED_EDGE ( 'NONE', *, *, #59941, .F. ) ;
#50773=ORIENTED_EDGE ( 'NONE', *, *, #32349, .T. ) ;
#50774=AXIS2_PLACEMENT_3D ( 'NONE', #31069, #70968, #21217 ) ;
#50775=DIRECTION ( 'NONE',  ( -4.274815082592931898E-19, -0.9999939076577903929, -0.003490651415223739937 ) ) ;
#50776=DIRECTION ( 'NONE',  ( -0.000000000000000000, -1.000000000000000000, -0.000000000000000000 ) ) ;
#50777=DIRECTION ( 'NONE',  ( 0.000000000000000000, 0.000000000000000000, 1.000000000000000000 ) ) ;
#50778=CARTESIAN_POINT ( 'NONE',  ( 10.84999999999990905, 2.500000000000000000, 2.065063509461097624 ) ) ;
#50779=VERTEX_POINT ( 'NONE', #128549 ) ;
#50780=LINE ( 'NONE', #71704, #77384 ) ;
#50781=AXIS2_PLACEMENT_3D ( 'NONE', #124569, #85273, #76751 ) ;
#50782=ORIENTED_EDGE ( 'NONE', *, *, #79007, .F. ) ;
#50783=DIRECTION ( 'NONE',  ( 0.000000000000000000, 0.000000000000000000, 1.000000000000000000 ) ) ;
#50784=CIRCLE ( 'NONE', #42379, 0.06509327318403745899 ) ;
#50785=AXIS2_PLACEMENT_3D ( 'NONE', #54641, #23919, #65755 ) ;
#50786=ORIENTED_EDGE ( 'NONE', *, *, #13769, .T. ) ;
#50787=DIRECTION ( 'NONE',  ( 0.000000000000000000, 0.000000000000000000, -1.000000000000000000 ) ) ;
#50788=DIRECTION ( 'NONE',  ( 0.000000000000000000, 0.000000000000000000, -1.000000000000000000 ) ) ;
#50789=CARTESIAN_POINT ( 'NONE',  ( -4.150000000000025224, 12.50000000000000000, 2.922977105672686982 ) ) ;
#50790=EDGE_CURVE ( 'NONE', #71326, #122362, #38885, .T. ) ;
#50791=DIRECTION ( 'NONE',  ( -0.000000000000000000, -1.000000000000000000, -0.000000000000000000 ) ) ;
#50792=VECTOR ( 'NONE', #55680, 1000.000000000000000 ) ;
#50793=VERTEX_POINT ( 'NONE', #76202 ) ;
#50794=CIRCLE ( 'NONE', #6843, 0.06509327318403745899 ) ;
#50795=EDGE_CURVE ( 'NONE', #110101, #32791, #116113, .T. ) ;
#50796=VECTOR ( 'NONE', #11124, 1000.000000000000000 ) ;
#50797=DIRECTION ( 'NONE',  ( -4.274815082592931898E-19, -0.9999939076577903929, -0.003490651415223739937 ) ) ;
#50798=CONICAL_SURFACE ( 'NONE', #36225, 0.1000000000000002554, 0.003490658503988666988 ) ;
#50799=ADVANCED_FACE ( 'NONE', ( #37572 ), #18562, .T. ) ;
#50800=CARTESIAN_POINT ( 'NONE',  ( 8.149999999999920419, 2.500000000000000000, 6.148780366869520897 ) ) ;
#50801=ORIENTED_EDGE ( 'NONE', *, *, #49597, .T. ) ;
#50802=ORIENTED_EDGE ( 'NONE', *, *, #103649, .T. ) ;
#50803=ORIENTED_EDGE ( 'NONE', *, *, #100077, .T. ) ;
#50804=CARTESIAN_POINT ( 'NONE',  ( -2.700000000000029932, 12.50000000000000000, -0.4115034346978156399 ) ) ;
#50805=CARTESIAN_POINT ( 'NONE',  ( 6.049999999999934097, 2.500000000000000000, 6.248780366869521430 ) ) ;
#50806=DIRECTION ( 'NONE',  ( -0.000000000000000000, 1.000000000000000000, -0.000000000000000000 ) ) ;
#50807=CONICAL_SURFACE ( 'NONE', #48753, 0.09999999999999982514, 0.003490658503988666988 ) ;
#50808=LINE ( 'NONE', #20703, #55310 ) ;
#50809=EDGE_CURVE ( 'NONE', #114240, #78540, #98119, .T. ) ;
#50810=DIRECTION ( 'NONE',  ( 0.000000000000000000, 0.000000000000000000, -1.000000000000000000 ) ) ;
#50811=AXIS2_PLACEMENT_3D ( 'NONE', #26669, #106509, #78356 ) ;
#50812=CARTESIAN_POINT ( 'NONE',  ( -12.49999999999995914, 2.500000000000000000, -4.230127018922199333 ) ) ;
#50813=CIRCLE ( 'NONE', #111425, 0.1000000000000002554 ) ;
#50814=DIRECTION ( 'NONE',  ( 0.000000000000000000, -0.000000000000000000, 1.000000000000000000 ) ) ;
#50815=AXIS2_PLACEMENT_3D ( 'NONE', #126292, #26796, #66707 ) ;
#50816=AXIS2_PLACEMENT_3D ( 'NONE', #78469, #98079, #126908 ) ;
#50817=DIRECTION ( 'NONE',  ( 0.000000000000000000, 0.000000000000000000, 1.000000000000000000 ) ) ;
#50818=AXIS2_PLACEMENT_3D ( 'NONE', #71175, #111077, #41744 ) ;
#50819=EDGE_LOOP ( 'NONE', ( #89270, #67018 ) ) ;
#50820=CARTESIAN_POINT ( 'NONE',  ( -2.900000000000029221, 2.500000000000000000, 0.09999999999999772959 ) ) ;
#50821=DIRECTION ( 'NONE',  ( 0.000000000000000000, 0.000000000000000000, -1.000000000000000000 ) ) ;
#50822=ADVANCED_FACE ( 'NONE', ( #108229 ), #39665, .T. ) ;
#50823=CARTESIAN_POINT ( 'NONE',  ( 12.09999999999990550, 2.500000000000000000, 3.737306695894644371 ) ) ;
#50824=CARTESIAN_POINT ( 'NONE',  ( 2.049999999999950084, 12.50000000000000000, 2.165063509461097713 ) ) ;
#50825=EDGE_LOOP ( 'NONE', ( #66153, #64028 ) ) ;
#50826=CARTESIAN_POINT ( 'NONE',  ( 10.39999999999991509, 2.500000000000000000, -0.6928203230275542523 ) ) ;
#50827=LINE ( 'NONE', #51480, #36557 ) ;
#50828=DIRECTION ( 'NONE',  ( 0.000000000000000000, 0.000000000000000000, 1.000000000000000000 ) ) ;
#50829=EDGE_LOOP ( 'NONE', ( #33905, #104539, #97309, #24364 ) ) ;
#50830=CONICAL_SURFACE ( 'NONE', #17447, 0.09999999999999982514, 0.003490658503988666988 ) ;
#50831=ORIENTED_EDGE ( 'NONE', *, *, #57877, .T. ) ;
#50832=DIRECTION ( 'NONE',  ( 0.000000000000000000, 0.000000000000000000, 1.000000000000000000 ) ) ;
#50833=VECTOR ( 'NONE', #34434, 1000.000000000000000 ) ;
#50834=EDGE_CURVE ( 'NONE', #65564, #102028, #46740, .T. ) ;
#50835=ORIENTED_EDGE ( 'NONE', *, *, #94932, .T. ) ;
#50836=AXIS2_PLACEMENT_3D ( 'NONE', #1927, #30777, #110599 ) ;
#50837=VERTEX_POINT ( 'NONE', #88595 ) ;
#50838=DIRECTION ( 'NONE',  ( 0.000000000000000000, 0.000000000000000000, 1.000000000000000000 ) ) ;
#50839=AXIS2_PLACEMENT_3D ( 'NONE', #52210, #122888, #123510 ) ;
#50840=CIRCLE ( 'NONE', #34118, 0.1000000000000002554 ) ;
#50841=DIRECTION ( 'NONE',  ( 0.000000000000000000, 0.000000000000000000, 1.000000000000000000 ) ) ;
#50842=LINE ( 'NONE', #31851, #63048 ) ;
#50844=AXIS2_PLACEMENT_3D ( 'NONE', #68848, #118584, #27616 ) ;
#50845=ORIENTED_EDGE ( 'NONE', *, *, #65381, .F. ) ;
#50846=CIRCLE ( 'NONE', #11109, 0.06509327318403745899 ) ;
#50848=PLANE ( 'NONE',  #25186 ) ;
#50849=CIRCLE ( 'NONE', #88487, 0.06509327318403745899 ) ;
#50850=ORIENTED_EDGE ( 'NONE', *, *, #39109, .T. ) ;
#50851=AXIS2_PLACEMENT_3D ( 'NONE', #108736, #59004, #98925 ) ;
#50852=DIRECTION ( 'NONE',  ( 0.000000000000000000, 0.000000000000000000, 1.000000000000000000 ) ) ;
#50853=EDGE_CURVE ( 'NONE', #54395, #87768, #22923, .T. ) ;
#50854=CARTESIAN_POINT ( 'NONE',  ( 17.01005371150556655, -1.931450858213975774, 5.528361852685534039 ) ) ;
#50855=CIRCLE ( 'NONE', #36199, 0.06509327318403745899 ) ;
#50856=ORIENTED_EDGE ( 'NONE', *, *, #16417, .F. ) ;
#50857=ORIENTED_EDGE ( 'NONE', *, *, #84894, .F. ) ;
#50858=ORIENTED_EDGE ( 'NONE', *, *, #99656, .T. ) ;
#50859=EDGE_LOOP ( 'NONE', ( #32205, #76214 ) ) ;
#50860=DIRECTION ( 'NONE',  ( -0.000000000000000000, -1.000000000000000000, -0.000000000000000000 ) ) ;
#50861=CARTESIAN_POINT ( 'NONE',  ( 14.66596005923860702, 1.500000000000160538, 7.515560522276493849 ) ) ;
#50862=LINE ( 'NONE', #12206, #27438 ) ;
#50863=FACE_BOUND ( 'NONE', #122431, .T. ) ;
#50864=LINE ( 'NONE', #95136, #20229 ) ;
#50866=LINE ( 'NONE', #61333, #113789 ) ;
#50867=DIRECTION ( 'NONE',  ( 0.000000000000000000, -0.9999939076577903929, 0.003490651415223739937 ) ) ;
#50868=AXIS2_PLACEMENT_3D ( 'NONE', #47963, #96389, #127798 ) ;
#50869=CARTESIAN_POINT ( 'NONE',  ( 3.099999999999945466, 2.500000000000000000, 0.3464101615137735735 ) ) ;
#50870=CARTESIAN_POINT ( 'NONE',  ( 4.149999999999941735, 2.500000000000000000, -2.857883832488653741 ) ) ;
#50871=DIRECTION ( 'NONE',  ( 0.000000000000000000, 0.000000000000000000, 1.000000000000000000 ) ) ;
#50872=VECTOR ( 'NONE', #24476, 1000.000000000000000 ) ;
#50874=CARTESIAN_POINT ( 'NONE',  ( -2.300000000000032685, 2.500000000000000000, -0.3464101615137783474 ) ) ;
#50875=EDGE_CURVE ( 'NONE', #11372, #118034, #27028, .T. ) ;
#50876=ORIENTED_EDGE ( 'NONE', *, *, #90766, .T. ) ;
#50878=VERTEX_POINT ( 'NONE', #47387 ) ;
#50880=ORIENTED_EDGE ( 'NONE', *, *, #29745, .T. ) ;
#50881=PLANE ( 'NONE',  #2116 ) ;
#50882=DIRECTION ( 'NONE',  ( 0.000000000000000000, 1.000000000000000000, 0.000000000000000000 ) ) ;
#50883=VERTEX_POINT ( 'NONE', #64118 ) ;
#50884=FACE_BOUND ( 'NONE', #39336, .T. ) ;
#50885=VECTOR ( 'NONE', #16146, 1000.000000000000000 ) ;
#50886=FACE_OUTER_BOUND ( 'NONE', #75572, .T. ) ;
#50887=AXIS2_PLACEMENT_3D ( 'NONE', #38378, #118847, #89395 ) ;
#50888=EDGE_CURVE ( 'NONE', #110619, #101819, #96063, .T. ) ;
#50889=AXIS2_PLACEMENT_3D ( 'NONE', #1080, #31838, #51490 ) ;
#50890=ORIENTED_EDGE ( 'NONE', *, *, #977, .F. ) ;
#50891=EDGE_CURVE ( 'NONE', #109714, #114322, #110802, .T. ) ;
#50892=CARTESIAN_POINT ( 'NONE',  ( 5.399999999999934630, 2.500000000000000000, 0.5928203230275495006 ) ) ;
#50893=DIRECTION ( 'NONE',  ( -4.274815082592931898E-19, -0.9999939076577903929, -0.003490651415223739937 ) ) ;
#50894=EDGE_CURVE ( 'NONE', #86833, #65792, #41709, .T. ) ;
#50895=CARTESIAN_POINT ( 'NONE',  ( 11.89999999999990443, 12.50000000000000000, -0.3464101615137782364 ) ) ;
#50896=ADVANCED_FACE ( 'NONE', ( #72191 ), #102341, .T. ) ;
#50897=DIRECTION ( 'NONE',  ( 0.000000000000000000, 0.000000000000000000, 1.000000000000000000 ) ) ;
#50898=CIRCLE ( 'NONE', #124047, 0.06509327318403745899 ) ;
#50899=EDGE_CURVE ( 'NONE', #120246, #71888, #16629, .T. ) ;
#50900=VERTEX_POINT ( 'NONE', #22455 ) ;
#50901=DIRECTION ( 'NONE',  ( -0.000000000000000000, -1.000000000000000000, -0.000000000000000000 ) ) ;
#50902=CIRCLE ( 'NONE', #67601, 0.1000000000000000472 ) ;
#50903=AXIS2_PLACEMENT_3D ( 'NONE', #25183, #35664, #36326 ) ;
#50904=AXIS2_PLACEMENT_3D ( 'NONE', #6299, #44978, #86152 ) ;
#50905=ORIENTED_EDGE ( 'NONE', *, *, #40290, .T. ) ;
#50906=EDGE_CURVE ( 'NONE', #87824, #9138, #857, .T. ) ;
#50907=VERTEX_POINT ( 'NONE', #40143 ) ;
#50908=CARTESIAN_POINT ( 'NONE',  ( -8.350000000000012079, 2.500000000000000000, 1.472243186433545459 ) ) ;
#50909=ADVANCED_FACE ( 'NONE', ( #61060 ), #129196, .T. ) ;
#50910=DIRECTION ( 'NONE',  ( 0.000000000000000000, 0.000000000000000000, 1.000000000000000000 ) ) ;
#50911=CIRCLE ( 'NONE', #19602, 0.06509327318403745899 ) ;
#50912=ORIENTED_EDGE ( 'NONE', *, *, #119469, .F. ) ;
#50913=EDGE_CURVE ( 'NONE', #113123, #116569, #125317, .T. ) ;
#50914=FACE_OUTER_BOUND ( 'NONE', #3512, .T. ) ;
#50915=EDGE_CURVE ( 'NONE', #86766, #23803, #106526, .T. ) ;
#50916=DIRECTION ( 'NONE',  ( 0.000000000000000000, 0.000000000000000000, 1.000000000000000000 ) ) ;
#50917=ADVANCED_FACE ( 'NONE', ( #11321 ), #70939, .T. ) ;
#50918=DIRECTION ( 'NONE',  ( 0.000000000000000000, -0.9999939076577903929, 0.003490651415223739937 ) ) ;
#50919=DIRECTION ( 'NONE',  ( 0.000000000000000000, 0.000000000000000000, 1.000000000000000000 ) ) ;
#50920=ORIENTED_EDGE ( 'NONE', *, *, #57723, .T. ) ;
#50921=DIRECTION ( 'NONE',  ( 0.000000000000000000, 0.000000000000000000, 1.000000000000000000 ) ) ;
#50922=EDGE_CURVE ( 'NONE', #99646, #55120, #52160, .T. ) ;
#50923=ORIENTED_EDGE ( 'NONE', *, *, #54052, .F. ) ;
#50925=ORIENTED_EDGE ( 'NONE', *, *, #5386, .T. ) ;
#50926=CARTESIAN_POINT ( 'NONE',  ( 14.59999999999989484, 2.500000000000000000, -0.1000000000000022815 ) ) ;
#50927=ORIENTED_EDGE ( 'NONE', *, *, #12632, .F. ) ;
#50928=FACE_OUTER_BOUND ( 'NONE', #98621, .T. ) ;
#50929=CARTESIAN_POINT ( 'NONE',  ( -12.29999999999999716, 2.500000000000000000, -3.983716857408423628 ) ) ;
#50930=CIRCLE ( 'NONE', #109404, 0.1000000000000000472 ) ;
#50931=DIRECTION ( 'NONE',  ( 0.000000000000000000, 0.000000000000000000, 1.000000000000000000 ) ) ;
#50932=CIRCLE ( 'NONE', #119873, 0.09999999999999999167 ) ;
#50933=PLANE ( 'NONE',  #57098 ) ;
#50934=DIRECTION ( 'NONE',  ( 0.000000000000000000, 1.000000000000000000, 0.000000000000000000 ) ) ;
#50935=EDGE_LOOP ( 'NONE', ( #87052, #89794 ) ) ;
#50936=ORIENTED_EDGE ( 'NONE', *, *, #97136, .F. ) ;
#50937=ORIENTED_EDGE ( 'NONE', *, *, #3808, .F. ) ;
#50938=DIRECTION ( 'NONE',  ( 0.000000000000000000, 0.000000000000000000, 1.000000000000000000 ) ) ;
#50939=CIRCLE ( 'NONE', #17550, 0.09999999999999999167 ) ;
#50940=AXIS2_PLACEMENT_3D ( 'NONE', #64003, #103930, #94740 ) ;
#50941=VECTOR ( 'NONE', #9672, 1000.000000000000000 ) ;
#50943=AXIS2_PLACEMENT_3D ( 'NONE', #98548, #107750, #77630 ) ;
#50944=AXIS2_PLACEMENT_3D ( 'NONE', #85256, #73488, #24403 ) ;
#50945=DIRECTION ( 'NONE',  ( 0.000000000000000000, 1.000000000000000000, 0.000000000000000000 ) ) ;
#50946=ORIENTED_EDGE ( 'NONE', *, *, #69141, .F. ) ;
#50947=ORIENTED_EDGE ( 'NONE', *, *, #38212, .T. ) ;
#50948=VERTEX_POINT ( 'NONE', #60448 ) ;
#50949=DIRECTION ( 'NONE',  ( 0.000000000000000000, -0.000000000000000000, 1.000000000000000000 ) ) ;
#50950=VERTEX_POINT ( 'NONE', #121923 ) ;
#50951=DIRECTION ( 'NONE',  ( -0.000000000000000000, -1.000000000000000000, -0.000000000000000000 ) ) ;
#50952=VECTOR ( 'NONE', #79802, 1000.000000000000000 ) ;
#50953=DIRECTION ( 'NONE',  ( 0.000000000000000000, -0.000000000000000000, 1.000000000000000000 ) ) ;
#50954=B_SPLINE_CURVE_WITH_KNOTS ( 'NONE', 3,
 ( #76618, #115888, #116529, #7209 ),
 .UNSPECIFIED., .F., .F.,
 ( 4, 4 ),
 ( 4.336808689942017736E-19, 0.002128161363186974360 ),
 .UNSPECIFIED. ) ;
#50955=CARTESIAN_POINT ( 'NONE',  ( 12.69999999999990159, 2.500000000000000000, 4.676537180435972552 ) ) ;
#50956=CARTESIAN_POINT ( 'NONE',  ( -10.85000000000000142, 2.500000000000000000, -1.372243186433546036 ) ) ;
#50957=CARTESIAN_POINT ( 'NONE',  ( -3.350000000000028955, 2.500000000000000000, -2.165063509461101710 ) ) ;
#50958=CARTESIAN_POINT ( 'NONE',  ( -7.900000000000011013, 2.500000000000000000, 5.022947341949748790 ) ) ;
#50959=VECTOR ( 'NONE', #7803, 1000.000000000000000 ) ;
#50960=CARTESIAN_POINT ( 'NONE',  ( -7.500000000000001776, -1.500000000000000000, -9.999999999999998224 ) ) ;
#50961=ORIENTED_EDGE ( 'NONE', *, *, #52420, .F. ) ;
#50962=ORIENTED_EDGE ( 'NONE', *, *, #43683, .F. ) ;
#50963=EDGE_CURVE ( 'NONE', #31381, #74338, #89803, .T. ) ;
#50964=CARTESIAN_POINT ( 'NONE',  ( 6.849999999999929479, 12.50000000000000000, 6.906693963081109722 ) ) ;
#50965=CARTESIAN_POINT ( 'NONE',  ( 3.149999999999946176, 2.500000000000000000, -6.941600689897077459 ) ) ;
#50966=EDGE_CURVE ( 'NONE', #30332, #15328, #114835, .T. ) ;
#50967=ORIENTED_EDGE ( 'NONE', *, *, #115485, .T. ) ;
#50969=ORIENTED_EDGE ( 'NONE', *, *, #90766, .F. ) ;
#50972=LINE ( 'NONE', #71897, #70866 ) ;
#50973=AXIS2_PLACEMENT_3D ( 'NONE', #49904, #91097, #38810 ) ;
#50974=DIRECTION ( 'NONE',  ( 0.000000000000000000, 0.000000000000000000, 1.000000000000000000 ) ) ;
#50975=EDGE_CURVE ( 'NONE', #116333, #22598, #10389, .T. ) ;
#50976=DIRECTION ( 'NONE',  ( 0.000000000000000000, 0.000000000000000000, 1.000000000000000000 ) ) ;
#50977=FACE_OUTER_BOUND ( 'NONE', #63293, .T. ) ;
#50978=CARTESIAN_POINT ( 'NONE',  ( 11.24999999999994316, 2.500000000000000000, -6.395190528383301931 ) ) ;
#50979=DIRECTION ( 'NONE',  ( -4.274815082592931898E-19, -0.9999939076577903929, -0.003490651415223739937 ) ) ;
#50980=AXIS2_PLACEMENT_3D ( 'NONE', #29275, #36526, #118931 ) ;
#50981=LINE ( 'NONE', #100068, #77140 ) ;
#50982=CIRCLE ( 'NONE', #124112, 0.06509327318403745899 ) ;
#50983=EDGE_LOOP ( 'NONE', ( #25276, #54769, #52726, #129225 ) ) ;
#50984=CIRCLE ( 'NONE', #71806, 0.06509327318403745899 ) ;
#50985=ORIENTED_EDGE ( 'NONE', *, *, #78090, .F. ) ;
#50986=EDGE_LOOP ( 'NONE', ( #114428, #56857, #685, #23720 ) ) ;
#50987=ORIENTED_EDGE ( 'NONE', *, *, #8890, .T. ) ;
#50988=ORIENTED_EDGE ( 'NONE', *, *, #2043, .F. ) ;
#50989=CIRCLE ( 'NONE', #119925, 0.06509327318403745899 ) ;
#50990=PLANE ( 'NONE',  #115313 ) ;
#50992=CIRCLE ( 'NONE', #76008, 0.09999999999999982514 ) ;
#50993=CIRCLE ( 'NONE', #22074, 0.09999999999999999167 ) ;
#50994=ORIENTED_EDGE ( 'NONE', *, *, #107947, .F. ) ;
#50995=CARTESIAN_POINT ( 'NONE',  ( -1.650000000000034328, 12.50000000000000000, -7.122917578226816815 ) ) ;
#50996=DIRECTION ( 'NONE',  ( -0.000000000000000000, 1.000000000000000000, -0.000000000000000000 ) ) ;
#50997=DIRECTION ( 'NONE',  ( 0.000000000000000000, -0.000000000000000000, 1.000000000000000000 ) ) ;
#50998=LINE ( 'NONE', #121008, #7730 ) ;
#50999=ORIENTED_EDGE ( 'NONE', *, *, #11975, .T. ) ;
#51000=LINE ( 'NONE', #1236, #101829 ) ;
#51001=AXIS2_PLACEMENT_3D ( 'NONE', #120138, #19335, #80217 ) ;
#51002=DIRECTION ( 'NONE',  ( 0.000000000000000000, 0.000000000000000000, -1.000000000000000000 ) ) ;
#51003=EDGE_CURVE ( 'NONE', #46382, #88884, #29192, .T. ) ;
#51004=ORIENTED_EDGE ( 'NONE', *, *, #126689, .T. ) ;
#51005=AXIS2_PLACEMENT_3D ( 'NONE', #97058, #114117, #15246 ) ;
#51006=CIRCLE ( 'NONE', #88643, 0.1000000000000002554 ) ;
#51007=CIRCLE ( 'NONE', #126303, 0.09999999999999999167 ) ;
#51008=ORIENTED_EDGE ( 'NONE', *, *, #7883, .F. ) ;
#51009=ORIENTED_EDGE ( 'NONE', *, *, #57740, .T. ) ;
#51010=EDGE_LOOP ( 'NONE', ( #103521, #50124 ) ) ;
#51011=DIRECTION ( 'NONE',  ( -0.000000000000000000, -1.000000000000000000, -0.000000000000000000 ) ) ;
#51012=AXIS2_PLACEMENT_3D ( 'NONE', #49950, #29009, #128519 ) ;
#51013=FACE_OUTER_BOUND ( 'NONE', #72940, .T. ) ;
#51014=FACE_OUTER_BOUND ( 'NONE', #105259, .T. ) ;
#51015=CIRCLE ( 'NONE', #99020, 0.1000000000000002554 ) ;
#51016=CARTESIAN_POINT ( 'NONE',  ( -3.150000000000032330, 12.50000000000000000, -6.083687093685488989 ) ) ;
#51017=ADVANCED_FACE ( 'NONE', ( #111440 ), #6169, .T. ) ;
#51018=ORIENTED_EDGE ( 'NONE', *, *, #94895, .T. ) ;
#51019=FACE_OUTER_BOUND ( 'NONE', #50295, .T. ) ;
#51020=PLANE ( 'NONE',  #22570 ) ;
#51021=DIRECTION ( 'NONE',  ( 0.000000000000000000, 0.000000000000000000, 1.000000000000000000 ) ) ;
#51022=CARTESIAN_POINT ( 'NONE',  ( 21.24754738303277435, -0.7337760880902347571, 4.182111650399361835 ) ) ;
#51023=EDGE_CURVE ( 'NONE', #67661, #108498, #64670, .T. ) ;
#51024=ORIENTED_EDGE ( 'NONE', *, *, #34477, .F. ) ;
#51025=ORIENTED_EDGE ( 'NONE', *, *, #64064, .F. ) ;
#51026=VERTEX_POINT ( 'NONE', #61732 ) ;
#51027=CARTESIAN_POINT ( 'NONE',  ( 0.8499999999999553468, 12.50000000000000000, -2.230156782645139391 ) ) ;
#51028=CIRCLE ( 'NONE', #67721, 0.06509327318403745899 ) ;
#51029=CONICAL_SURFACE ( 'NONE', #80264, 0.09999999999999982514, 0.003490658503988666988 ) ;
#51030=ADVANCED_FACE ( 'NONE', ( #91817 ), #114926, .T. ) ;
#51032=FACE_BOUND ( 'NONE', #52208, .T. ) ;
#51033=CARTESIAN_POINT ( 'NONE',  ( -15.39999999999998082, 2.500000000000000000, 0.6928203230275518099 ) ) ;
#51035=DIRECTION ( 'NONE',  ( 0.000000000000000000, 0.000000000000000000, 1.000000000000000000 ) ) ;
#51036=AXIS2_PLACEMENT_3D ( 'NONE', #54527, #103656, #22534 ) ;
#51037=AXIS2_PLACEMENT_3D ( 'NONE', #22012, #70449, #39079 ) ;
#51038=AXIS2_PLACEMENT_3D ( 'NONE', #34365, #8569, #77331 ) ;
#51039=DIRECTION ( 'NONE',  ( 0.000000000000000000, 0.000000000000000000, 1.000000000000000000 ) ) ;
#51040=FACE_OUTER_BOUND ( 'NONE', #129232, .T. ) ;
#51041=CARTESIAN_POINT ( 'NONE',  ( -13.34999999999999076, 2.500000000000000000, -1.572243186433547990 ) ) ;
#51042=VERTEX_POINT ( 'NONE', #64757 ) ;
#51043=VECTOR ( 'NONE', #13630, 1000.000000000000000 ) ;
#51044=DIRECTION ( 'NONE',  ( -0.000000000000000000, 1.000000000000000000, -0.000000000000000000 ) ) ;
#51045=CONICAL_SURFACE ( 'NONE', #46833, 0.1000000000000002554, 0.003490658503988666988 ) ;
#51046=CONICAL_SURFACE ( 'NONE', #28043, 0.1000000000000002554, 0.003490658503988666988 ) ;
#51047=DIRECTION ( 'NONE',  ( 0.000000000000000000, 1.000000000000000000, 0.000000000000000000 ) ) ;
#51048=ORIENTED_EDGE ( 'NONE', *, *, #118642, .T. ) ;
#51049=VERTEX_POINT ( 'NONE', #44479 ) ;
#51050=AXIS2_PLACEMENT_3D ( 'NONE', #20216, #60159, #100066 ) ;
#51051=DIRECTION ( 'NONE',  ( -0.000000000000000000, -1.000000000000000000, -0.000000000000000000 ) ) ;
#51052=DIRECTION ( 'NONE',  ( 0.000000000000000000, 0.000000000000000000, 1.000000000000000000 ) ) ;
#51053=FACE_BOUND ( 'NONE', #128670, .T. ) ;
#51054=DIRECTION ( 'NONE',  ( 0.000000000000000000, 0.000000000000000000, -1.000000000000000000 ) ) ;
#51055=EDGE_CURVE ( 'NONE', #50102, #41939, #126919, .T. ) ;
#51056=CARTESIAN_POINT ( 'NONE',  ( -2.950000000000029932, 2.500000000000000000, 2.065063509461097624 ) ) ;
#51057=ORIENTED_EDGE ( 'NONE', *, *, #74151, .T. ) ;
#51058=DIRECTION ( 'NONE',  ( 0.000000000000000000, -0.9999939076577903929, 0.003490651415223739937 ) ) ;
#51059=EDGE_CURVE ( 'NONE', #118212, #123047, #18785, .T. ) ;
#51061=ADVANCED_FACE ( 'NONE', ( #56223 ), #104471, .T. ) ;
#51063=ORIENTED_EDGE ( 'NONE', *, *, #66247, .F. ) ;
#51064=DIRECTION ( 'NONE',  ( -4.274815082592931898E-19, -0.9999939076577903929, -0.003490651415223739937 ) ) ;
#51065=PLANE ( 'NONE',  #70041 ) ;
#51066=ADVANCED_FACE ( 'NONE', ( #106614 ), #123355, .T. ) ;
#51067=EDGE_CURVE ( 'NONE', #22544, #93141, #14577, .T. ) ;
#51068=FACE_OUTER_BOUND ( 'NONE', #92278, .T. ) ;
#51069=ADVANCED_FACE ( 'NONE', ( #77167 ), #66690, .T. ) ;
#51070=CARTESIAN_POINT ( 'NONE',  ( -9.600000000000008527, 12.50000000000000000, -4.395220292106235327 ) ) ;
#51071=CIRCLE ( 'NONE', #44810, 0.06509327318403745899 ) ;
#51072=VERTEX_POINT ( 'NONE', #104673 ) ;
#51073=DIRECTION ( 'NONE',  ( 0.000000000000000000, 0.000000000000000000, -1.000000000000000000 ) ) ;
#51074=EDGE_CURVE ( 'NONE', #84952, #101891, #116431, .T. ) ;
#51075=FACE_OUTER_BOUND ( 'NONE', #34488, .T. ) ;
#51077=ORIENTED_EDGE ( 'NONE', *, *, #103963, .T. ) ;
#51078=ORIENTED_EDGE ( 'NONE', *, *, #89977, .F. ) ;
#51079=EDGE_CURVE ( 'NONE', #15576, #102929, #117068, .T. ) ;
#51080=DIRECTION ( 'NONE',  ( 0.000000000000000000, 0.000000000000000000, 1.000000000000000000 ) ) ;
#51081=EDGE_CURVE ( 'NONE', #87216, #120954, #79453, .T. ) ;
#51082=ORIENTED_EDGE ( 'NONE', *, *, #5051, .T. ) ;
#51083=CARTESIAN_POINT ( 'NONE',  ( -12.49999999999999467, 2.500000000000000000, -3.737306695894647035 ) ) ;
#51084=DIRECTION ( 'NONE',  ( 0.000000000000000000, 1.000000000000000000, 0.000000000000000000 ) ) ;
#51085=CIRCLE ( 'NONE', #82475, 0.1000000000000002554 ) ;
#51086=CARTESIAN_POINT ( 'NONE',  ( -5.200000000000022382, 12.50000000000000000, 4.676537180435972552 ) ) ;
#51087=ORIENTED_EDGE ( 'NONE', *, *, #91845, .T. ) ;
#51088=DIRECTION ( 'NONE',  ( -0.000000000000000000, -1.000000000000000000, -0.000000000000000000 ) ) ;
#51089=DIRECTION ( 'NONE',  ( 0.000000000000000000, 1.000000000000000000, 0.000000000000000000 ) ) ;
#51090=LINE ( 'NONE', #90996, #82035 ) ;
#51091=DIRECTION ( 'NONE',  ( -4.274815082592931898E-19, -0.9999939076577903929, -0.003490651415223739937 ) ) ;
#51092=CARTESIAN_POINT ( 'NONE',  ( -7.900000000000014566, 2.500000000000000000, -0.1000000000000022815 ) ) ;
#51093=DIRECTION ( 'NONE',  ( -0.000000000000000000, -1.000000000000000000, -0.000000000000000000 ) ) ;
#51094=EDGE_LOOP ( 'NONE', ( #52132, #76579, #36459, #53788 ) ) ;
#51095=VERTEX_POINT ( 'NONE', #47075 ) ;
#51096=DIRECTION ( 'NONE',  ( 0.000000000000000000, -0.9999939076577903929, 0.003490651415223739937 ) ) ;
#51097=VECTOR ( 'NONE', #100905, 1000.000000000000000 ) ;
#51098=ORIENTED_EDGE ( 'NONE', *, *, #69954, .T. ) ;
#51099=VECTOR ( 'NONE', #93049, 1000.000000000000000 ) ;
#51100=PLANE ( 'NONE',  #122462 ) ;
#51101=ORIENTED_EDGE ( 'NONE', *, *, #739, .T. ) ;
#51102=ORIENTED_EDGE ( 'NONE', *, *, #50790, .F. ) ;
#51103=VERTEX_POINT ( 'NONE', #45139 ) ;
#51104=AXIS2_PLACEMENT_3D ( 'NONE', #53155, #92420, #10615 ) ;
#51105=DIRECTION ( 'NONE',  ( 0.000000000000000000, 0.000000000000000000, -1.000000000000000000 ) ) ;
#51106=VECTOR ( 'NONE', #97380, 1000.000000000000000 ) ;
#51107=DIRECTION ( 'NONE',  ( 0.000000000000000000, 1.000000000000000000, 0.000000000000000000 ) ) ;
#51108=DIRECTION ( 'NONE',  ( 0.000000000000000000, 0.000000000000000000, -1.000000000000000000 ) ) ;
#51109=DIRECTION ( 'NONE',  ( 0.000000000000000000, 0.000000000000000000, 1.000000000000000000 ) ) ;
#51110=CARTESIAN_POINT ( 'NONE',  ( -5.650000000000023448, 2.500000000000000000, -6.248780366869526759 ) ) ;
#51111=DIRECTION ( 'NONE',  ( 0.000000000000000000, 1.000000000000000000, 0.000000000000000000 ) ) ;
#51112=DIRECTION ( 'NONE',  ( -0.000000000000000000, 1.000000000000000000, -0.000000000000000000 ) ) ;
#51113=CARTESIAN_POINT ( 'NONE',  ( 16.55874544816229488, 0.4845305829427787869, -6.091953208798931207 ) ) ;
#51114=CARTESIAN_POINT ( 'NONE',  ( -7.100000000000018296, 12.50000000000000000, -2.385244779468109755E-15 ) ) ;
#51115=EDGE_LOOP ( 'NONE', ( #70806, #9892 ) ) ;
#51116=ADVANCED_FACE ( 'NONE', ( #124337 ), #96156, .T. ) ;
#51117=AXIS2_PLACEMENT_3D ( 'NONE', #82524, #122440, #15018 ) ;
#51118=VECTOR ( 'NONE', #64637, 1000.000000000000000 ) ;
#51119=EDGE_CURVE ( 'NONE', #66361, #73062, #83561, .T. ) ;
#51120=LINE ( 'NONE', #99576, #67398 ) ;
#51121=VECTOR ( 'NONE', #69127, 1000.000000000000000 ) ;
#51122=CONICAL_SURFACE ( 'NONE', #115847, 0.1000000000000002554, 0.003490658503988666988 ) ;
#51123=ORIENTED_EDGE ( 'NONE', *, *, #77357, .T. ) ;
#51124=EDGE_LOOP ( 'NONE', ( #96449, #102003, #66129, #57020 ) ) ;
#51126=CARTESIAN_POINT ( 'NONE',  ( 3.749999999999940492, 12.50000000000000000, 5.802370205355744659 ) ) ;
#51127=AXIS2_PLACEMENT_3D ( 'NONE', #90195, #100043, #18888 ) ;
#51128=DIRECTION ( 'NONE',  ( 0.000000000000000000, 0.000000000000000000, -1.000000000000000000 ) ) ;
#51129=VECTOR ( 'NONE', #70702, 1000.000000000000000 ) ;
#51130=AXIS2_PLACEMENT_3D ( 'NONE', #60619, #103098, #93284 ) ;
#51131=CARTESIAN_POINT ( 'NONE',  ( 6.649999999999931077, 12.50000000000000000, -6.430097255199264339 ) ) ;
#51132=DIRECTION ( 'NONE',  ( 0.000000000000000000, 0.000000000000000000, -1.000000000000000000 ) ) ;
#51133=DIRECTION ( 'NONE',  ( 0.000000000000000000, -0.000000000000000000, 1.000000000000000000 ) ) ;
#51134=VERTEX_POINT ( 'NONE', #14991 ) ;
#51136=EDGE_LOOP ( 'NONE', ( #48215, #46041, #99396, #2342 ) ) ;
#51137=VECTOR ( 'NONE', #51064, 1000.000000000000000 ) ;
#51138=VERTEX_POINT ( 'NONE', #66049 ) ;
#51139=CARTESIAN_POINT ( 'NONE',  ( -14.14999999999998614, 2.500000000000000000, 1.472243186433549456 ) ) ;
#51140=ORIENTED_EDGE ( 'NONE', *, *, #62204, .F. ) ;
#51141=CIRCLE ( 'NONE', #124290, 0.06509327318403745899 ) ;
#51142=VERTEX_POINT ( 'NONE', #95521 ) ;
#51143=DIRECTION ( 'NONE',  ( 0.000000000000000000, 0.000000000000000000, 1.000000000000000000 ) ) ;
#51144=DIRECTION ( 'NONE',  ( -0.000000000000000000, -1.000000000000000000, -0.000000000000000000 ) ) ;
#51145=DIRECTION ( 'NONE',  ( 0.000000000000000000, -0.9999939076577903929, 0.003490651415223739937 ) ) ;
#51146=CARTESIAN_POINT ( 'NONE',  ( 10.19999999999991580, 12.50000000000000000, -0.3464101615137783474 ) ) ;
#51147=DIRECTION ( 'NONE',  ( -0.000000000000000000, -1.000000000000000000, -0.000000000000000000 ) ) ;
#51148=VERTEX_POINT ( 'NONE', #94871 ) ;
#51149=CARTESIAN_POINT ( 'NONE',  ( -5.850000000000022737, 12.50000000000000000, -2.099970236277064473 ) ) ;
#51150=FACE_OUTER_BOUND ( 'NONE', #109236, .T. ) ;
#51151=LINE ( 'NONE', #91060, #66632 ) ;
#51152=PLANE ( 'NONE',  #28486 ) ;
#51153=AXIS2_PLACEMENT_3D ( 'NONE', #93791, #113425, #33588 ) ;
#51154=DIRECTION ( 'NONE',  ( 0.000000000000000000, 1.000000000000000000, 0.000000000000000000 ) ) ;
#51155=EDGE_CURVE ( 'NONE', #2020, #2451, #46404, .T. ) ;
#51156=VERTEX_POINT ( 'NONE', #5184 ) ;
#51157=ORIENTED_EDGE ( 'NONE', *, *, #103558, .T. ) ;
#51158=ORIENTED_EDGE ( 'NONE', *, *, #79012, .F. ) ;
#51159=DIRECTION ( 'NONE',  ( 0.000000000000000000, 1.000000000000000000, 0.000000000000000000 ) ) ;
#51160=VERTEX_POINT ( 'NONE', #105981 ) ;
#51161=CONICAL_SURFACE ( 'NONE', #95070, 0.09999999999999982514, 0.003490658503988666988 ) ;
#51162=LINE ( 'NONE', #91070, #123933 ) ;
#51163=DIRECTION ( 'NONE',  ( 0.000000000000000000, 1.000000000000000000, 0.000000000000000000 ) ) ;
#51164=EDGE_CURVE ( 'NONE', #58918, #112146, #81504, .T. ) ;
#51165=AXIS2_PLACEMENT_3D ( 'NONE', #20920, #19636, #623 ) ;
#51166=EDGE_CURVE ( 'NONE', #76721, #115200, #100276, .T. ) ;
#51167=ORIENTED_EDGE ( 'NONE', *, *, #10641, .T. ) ;
#51168=CARTESIAN_POINT ( 'NONE',  ( -7.900000000000011013, 2.500000000000000000, 3.637306695894644726 ) ) ;
#51169=CARTESIAN_POINT ( 'NONE',  ( -9.600000000000006750, 12.50000000000000000, 3.637306695894644726 ) ) ;
#51170=PLANE ( 'NONE',  #191 ) ;
#51171=EDGE_CURVE ( 'NONE', #122705, #41669, #48056, .T. ) ;
#51172=DIRECTION ( 'NONE',  ( 0.000000000000000000, 1.000000000000000000, 0.000000000000000000 ) ) ;
#51173=AXIS2_PLACEMENT_3D ( 'NONE', #106845, #15894, #36849 ) ;
#51174=CARTESIAN_POINT ( 'NONE',  ( -10.80000000000000071, 12.50000000000000000, 4.330127018922196314 ) ) ;
#51175=EDGE_CURVE ( 'NONE', #51588, #125598, #89898, .T. ) ;
#51176=CONICAL_SURFACE ( 'NONE', #7223, 0.1000000000000002554, 0.003490658503988666988 ) ;
#51177=ORIENTED_EDGE ( 'NONE', *, *, #28870, .F. ) ;
#51178=VERTEX_POINT ( 'NONE', #19529 ) ;
#51180=CARTESIAN_POINT ( 'NONE',  ( 23.99341564996507259, 2.839174804732068846, -2.508498394836132572 ) ) ;
#51181=CARTESIAN_POINT ( 'NONE',  ( -9.550000000000006040, 2.500000000000000000, -2.265063509461101798 ) ) ;
#51182=DIRECTION ( 'NONE',  ( 0.000000000000000000, 0.000000000000000000, 1.000000000000000000 ) ) ;
#51183=CARTESIAN_POINT ( 'NONE',  ( 3.149999999999944400, 2.500000000000000000, 2.511473670974873507 ) ) ;
#51184=VERTEX_POINT ( 'NONE', #117709 ) ;
#51185=VECTOR ( 'NONE', #31114, 1000.000000000000000 ) ;
#51186=VECTOR ( 'NONE', #98860, 1000.000000000000000 ) ;
#51187=ORIENTED_EDGE ( 'NONE', *, *, #111788, .F. ) ;
#51188=CARTESIAN_POINT ( 'NONE',  ( -0.4000000000000331624, 12.50000000000000000, 0.000000000000000000 ) ) ;
#51189=CARTESIAN_POINT ( 'NONE',  ( 7.499999999999925393, 12.50000000000000000, -3.637306695894650055 ) ) ;
#51190=FACE_OUTER_BOUND ( 'NONE', #122563, .T. ) ;
#51192=ORIENTED_EDGE ( 'NONE', *, *, #92293, .T. ) ;
#51193=LINE ( 'NONE', #30911, #28097 ) ;
#51194=DIRECTION ( 'NONE',  ( -0.000000000000000000, 1.000000000000000000, -0.000000000000000000 ) ) ;
#51196=DIRECTION ( 'NONE',  ( 0.000000000000000000, -0.9999939076577903929, 0.003490651415223739937 ) ) ;
#51197=ORIENTED_EDGE ( 'NONE', *, *, #51344, .T. ) ;
#51198=CARTESIAN_POINT ( 'NONE',  ( -9.150000000000009237, 12.50000000000000000, 2.857883832488649301 ) ) ;
#51199=VERTEX_POINT ( 'NONE', #20178 ) ;
#51200=ADVANCED_FACE ( 'NONE', ( #79115 ), #28071, .T. ) ;
#51201=CIRCLE ( 'NONE', #63718, 0.1000000000000002554 ) ;
#51202=EDGE_LOOP ( 'NONE', ( #101073, #66776 ) ) ;
#51203=CARTESIAN_POINT ( 'NONE',  ( -12.89999999999999147, 12.50000000000000000, 1.843143693225357538E-15 ) ) ;
#51204=DIRECTION ( 'NONE',  ( -0.000000000000000000, -1.000000000000000000, -0.000000000000000000 ) ) ;
#51205=CONICAL_SURFACE ( 'NONE', #128483, 0.09999999999999982514, 0.003490658503988666988 ) ;
#51206=CIRCLE ( 'NONE', #7262, 0.09999999999999982514 ) ;
#51207=AXIS2_PLACEMENT_3D ( 'NONE', #129338, #102276, #93743 ) ;
#51208=EDGE_LOOP ( 'NONE', ( #5587, #39719, #91459, #105087 ) ) ;
#51209=ORIENTED_EDGE ( 'NONE', *, *, #33794, .T. ) ;
#51211=LINE ( 'NONE', #69534, #3874 ) ;
#51212=DIRECTION ( 'NONE',  ( -4.274815082592931898E-19, -0.9999939076577903929, -0.003490651415223739937 ) ) ;
#51213=EDGE_LOOP ( 'NONE', ( #21528, #3785 ) ) ;
#51214=EDGE_CURVE ( 'NONE', #16035, #52780, #107911, .T. ) ;
#51216=CIRCLE ( 'NONE', #9443, 0.06509327318403745899 ) ;
#51217=VECTOR ( 'NONE', #117400, 1000.000000000000000 ) ;
#51218=DIRECTION ( 'NONE',  ( 0.000000000000000000, 1.000000000000000000, 0.000000000000000000 ) ) ;
#51219=CARTESIAN_POINT ( 'NONE',  ( 6.049999999999934097, 2.500000000000000000, -2.411473670974877859 ) ) ;
#51220=PLANE ( 'NONE',  #126176 ) ;
#51221=EDGE_CURVE ( 'NONE', #3072, #84759, #90184, .T. ) ;
#51222=AXIS2_PLACEMENT_3D ( 'NONE', #65943, #56746, #27962 ) ;
#51223=CARTESIAN_POINT ( 'NONE',  ( -5.400000000000023448, 2.500000000000000000, -5.122947341949753763 ) ) ;
#51224=PLANE ( 'NONE',  #65178 ) ;
#51225=EDGE_CURVE ( 'NONE', #101891, #78289, #68971, .T. ) ;
#51226=EDGE_CURVE ( 'NONE', #118876, #97854, #83654, .T. ) ;
#51227=CIRCLE ( 'NONE', #124378, 0.1000000000000000472 ) ;
#51228=AXIS2_PLACEMENT_3D ( 'NONE', #116725, #65700, #46073 ) ;
#51229=ORIENTED_EDGE ( 'NONE', *, *, #20560, .T. ) ;
#51230=ORIENTED_EDGE ( 'NONE', *, *, #24188, .F. ) ;
#51231=DIRECTION ( 'NONE',  ( 0.000000000000000000, 0.000000000000000000, 1.000000000000000000 ) ) ;
#51232=EDGE_CURVE ( 'NONE', #48128, #78911, #12524, .T. ) ;
#51233=ORIENTED_EDGE ( 'NONE', *, *, #86638, .F. ) ;
#51234=DIRECTION ( 'NONE',  ( -4.274815082592931898E-19, -0.9999939076577903929, -0.003490651415223739937 ) ) ;
#51235=DIRECTION ( 'NONE',  ( 0.000000000000000000, 1.000000000000000000, 0.000000000000000000 ) ) ;
#51236=CIRCLE ( 'NONE', #90924, 0.1000000000000000472 ) ;
#51237=DIRECTION ( 'NONE',  ( -0.000000000000000000, -1.000000000000000000, -0.000000000000000000 ) ) ;
#51238=ORIENTED_EDGE ( 'NONE', *, *, #72895, .T. ) ;
#51239=ORIENTED_EDGE ( 'NONE', *, *, #70676, .T. ) ;
#51240=FACE_BOUND ( 'NONE', #8317, .T. ) ;
#51241=ORIENTED_EDGE ( 'NONE', *, *, #32552, .F. ) ;
#51242=DIRECTION ( 'NONE',  ( 0.000000000000000000, 0.000000000000000000, -1.000000000000000000 ) ) ;
#51243=FACE_OUTER_BOUND ( 'NONE', #26665, .T. ) ;
#51244=EDGE_CURVE ( 'NONE', #36298, #126837, #94009, .T. ) ;
#51246=LINE ( 'NONE', #46880, #24251 ) ;
#51247=ADVANCED_FACE ( 'NONE', ( #88249 ), #29274, .T. ) ;
#51248=CARTESIAN_POINT ( 'NONE',  ( -5.850000000000021849, 2.500000000000000000, -5.802370205355749988 ) ) ;
#51249=DIRECTION ( 'NONE',  ( 0.000000000000000000, 0.000000000000000000, -1.000000000000000000 ) ) ;
#51250=DIRECTION ( 'NONE',  ( 0.000000000000000000, -1.000000000000000000, 0.000000000000000000 ) ) ;
#51251=DIRECTION ( 'NONE',  ( -0.000000000000000000, 1.000000000000000000, -0.000000000000000000 ) ) ;
#51252=DIRECTION ( 'NONE',  ( 0.000000000000000000, 0.000000000000000000, -1.000000000000000000 ) ) ;
#51253=CARTESIAN_POINT ( 'NONE',  ( -0.2000000000000408673, 2.500000000000000000, -4.083716857408426826 ) ) ;
#51254=AXIS2_PLACEMENT_3D ( 'NONE', #125263, #15931, #25769 ) ;
#51255=DIRECTION ( 'NONE',  ( -0.000000000000000000, 1.000000000000000000, -0.000000000000000000 ) ) ;
#51256=VERTEX_POINT ( 'NONE', #128211 ) ;
#51257=ORIENTED_EDGE ( 'NONE', *, *, #17539, .F. ) ;
#51258=ORIENTED_EDGE ( 'NONE', *, *, #40833, .F. ) ;
#51259=EDGE_LOOP ( 'NONE', ( #96577, #83489, #120165, #77060 ) ) ;
#51260=DIRECTION ( 'NONE',  ( 0.000000000000000000, 0.000000000000000000, 1.000000000000000000 ) ) ;
#51261=DIRECTION ( 'NONE',  ( 0.000000000000000000, -0.000000000000000000, 1.000000000000000000 ) ) ;
#51262=ORIENTED_EDGE ( 'NONE', *, *, #26531, .T. ) ;
#51263=ORIENTED_EDGE ( 'NONE', *, *, #11711, .T. ) ;
#51264=EDGE_LOOP ( 'NONE', ( #69406, #77941, #87327, #104455 ) ) ;
#51265=CARTESIAN_POINT ( 'NONE',  ( -12.69999999999999218, 2.500000000000000000, -0.3464101615137741286 ) ) ;
#51266=CIRCLE ( 'NONE', #111884, 0.1000000000000002554 ) ;
#51267=AXIS2_PLACEMENT_3D ( 'NONE', #79679, #38498, #30605 ) ;
#51268=CARTESIAN_POINT ( 'NONE',  ( 0.8499999999999536815, 2.500000000000000000, 5.802370205355744659 ) ) ;
#51269=CARTESIAN_POINT ( 'NONE',  ( 5.849999999999933920, 2.500000000000000000, 5.802370205355744659 ) ) ;
#51270=CARTESIAN_POINT ( 'NONE',  ( 12.09999999999990195, 2.500000000000000000, 0.6928203230275494784 ) ) ;
#51271=DIRECTION ( 'NONE',  ( 0.000000000000000000, 1.000000000000000000, 0.000000000000000000 ) ) ;
#51272=PLANE ( 'NONE',  #7949 ) ;
#51273=DIRECTION ( 'NONE',  ( -0.000000000000000000, -1.000000000000000000, -0.000000000000000000 ) ) ;
#51274=EDGE_CURVE ( 'NONE', #6262, #31484, #37595, .T. ) ;
#51275=EDGE_LOOP ( 'NONE', ( #128848, #43541, #92548, #92536 ) ) ;
#51276=CARTESIAN_POINT ( 'NONE',  ( 2.899999999999944844, 2.500000000000000000, 3.637306695894644726 ) ) ;
#51277=ORIENTED_EDGE ( 'NONE', *, *, #120955, .T. ) ;
#51278=AXIS2_PLACEMENT_3D ( 'NONE', #124421, #83213, #93669 ) ;
#51280=EDGE_CURVE ( 'NONE', #19267, #114403, #64761, .T. ) ;
#51281=ORIENTED_EDGE ( 'NONE', *, *, #98565, .F. ) ;
#51282=CIRCLE ( 'NONE', #30352, 0.1000000000000002554 ) ;
#51283=DIRECTION ( 'NONE',  ( 0.000000000000000000, -0.9999939076577903929, 0.003490651415223739937 ) ) ;
#51285=ORIENTED_EDGE ( 'NONE', *, *, #17474, .T. ) ;
#51286=EDGE_LOOP ( 'NONE', ( #11085, #94339, #104498, #16934 ) ) ;
#51287=DIRECTION ( 'NONE',  ( 0.000000000000000000, 0.000000000000000000, 1.000000000000000000 ) ) ;
#51288=EDGE_CURVE ( 'NONE', #83267, #87429, #60128, .T. ) ;
#51289=DIRECTION ( 'NONE',  ( 0.000000000000000000, 0.000000000000000000, -1.000000000000000000 ) ) ;
#51290=CIRCLE ( 'NONE', #55474, 0.09999999999999982514 ) ;
#51291=CARTESIAN_POINT ( 'NONE',  ( 3.099999999999945466, 2.500000000000000000, 0.2464101615137735679 ) ) ;
#51292=CIRCLE ( 'NONE', #32425, 0.1000000000000002554 ) ;
#51293=CARTESIAN_POINT ( 'NONE',  ( -9.600000000000008527, 2.500000000000000000, 4.330127018922196314 ) ) ;
#51294=CARTESIAN_POINT ( 'NONE',  ( -10.65000000000000213, 2.500000000000000000, 1.918653347947321564 ) ) ;
#51295=DIRECTION ( 'NONE',  ( 0.000000000000000000, 0.000000000000000000, 1.000000000000000000 ) ) ;
#51296=DIRECTION ( 'NONE',  ( -0.000000000000000000, 1.000000000000000000, -0.000000000000000000 ) ) ;
#51297=VERTEX_POINT ( 'NONE', #17585 ) ;
#51298=DIRECTION ( 'NONE',  ( 0.000000000000000000, 0.000000000000000000, -1.000000000000000000 ) ) ;
#51299=EDGE_LOOP ( 'NONE', ( #29568, #78594 ) ) ;
#51300=DIRECTION ( 'NONE',  ( -0.000000000000000000, -1.000000000000000000, -0.000000000000000000 ) ) ;
#51301=LINE ( 'NONE', #92485, #21126 ) ;
#51302=VERTEX_POINT ( 'NONE', #87618 ) ;
#51303=DIRECTION ( 'NONE',  ( 0.000000000000000000, 0.000000000000000000, 1.000000000000000000 ) ) ;
#51304=DIRECTION ( 'NONE',  ( -0.000000000000000000, -1.000000000000000000, -0.000000000000000000 ) ) ;
#51305=AXIS2_PLACEMENT_3D ( 'NONE', #15657, #65415, #125616 ) ;
#51306=VERTEX_POINT ( 'NONE', #97445 ) ;
#51307=CIRCLE ( 'NONE', #97247, 0.06509327318403745899 ) ;
#51308=VECTOR ( 'NONE', #126640, 1000.000000000000000 ) ;
#51309=CARTESIAN_POINT ( 'NONE',  ( 9.149999999999920419, 12.50000000000000000, 2.857883832488649301 ) ) ;
#51310=VERTEX_POINT ( 'NONE', #127556 ) ;
#51311=CIRCLE ( 'NONE', #120569, 0.1000000000000002554 ) ;
#51312=VERTEX_POINT ( 'NONE', #37883 ) ;
#51313=DIRECTION ( 'NONE',  ( 0.000000000000000000, 0.000000000000000000, 1.000000000000000000 ) ) ;
#51314=DIRECTION ( 'NONE',  ( 0.000000000000000000, 0.000000000000000000, -1.000000000000000000 ) ) ;
#51316=CARTESIAN_POINT ( 'NONE',  ( 5.399999999999932854, 12.50000000000000000, 3.572213422710607489 ) ) ;
#51317=CIRCLE ( 'NONE', #82705, 0.06509327318403745899 ) ;
#51318=DIRECTION ( 'NONE',  ( -0.000000000000000000, 1.000000000000000000, -0.000000000000000000 ) ) ;
#51319=AXIS2_PLACEMENT_3D ( 'NONE', #79727, #77149, #128856 ) ;
#51320=ORIENTED_EDGE ( 'NONE', *, *, #30554, .F. ) ;
#51321=VECTOR ( 'NONE', #120660, 1000.000000000000000 ) ;
#51322=DIRECTION ( 'NONE',  ( -0.000000000000000000, -1.000000000000000000, -0.000000000000000000 ) ) ;
#51323=EDGE_LOOP ( 'NONE', ( #105535, #119911 ) ) ;
#51324=CONICAL_SURFACE ( 'NONE', #91015, 0.1000000000000000472, 0.003490658503988666988 ) ;
#51325=DIRECTION ( 'NONE',  ( 0.000000000000000000, 1.000000000000000000, 0.000000000000000000 ) ) ;
#51326=CARTESIAN_POINT ( 'NONE',  ( -6.250000000000015987, 12.50000000000000000, 5.867463478539781896 ) ) ;
#51327=VECTOR ( 'NONE', #3407, 1000.000000000000000 ) ;
#51328=EDGE_CURVE ( 'NONE', #18575, #104669, #77794, .T. ) ;
#51329=AXIS2_PLACEMENT_3D ( 'NONE', #112754, #23730, #114038 ) ;
#51330=CONICAL_SURFACE ( 'NONE', #36744, 0.09999999999999999167, 0.003490658503988666988 ) ;
#51331=EDGE_CURVE ( 'NONE', #89644, #25512, #54306, .T. ) ;
#51333=FACE_OUTER_BOUND ( 'NONE', #67176, .T. ) ;
#51334=DIRECTION ( 'NONE',  ( 0.000000000000000000, 1.000000000000000000, 0.000000000000000000 ) ) ;
#51335=CARTESIAN_POINT ( 'NONE',  ( 3.349999999999945466, 2.500000000000000000, -7.188010851410854052 ) ) ;
#51336=EDGE_CURVE ( 'NONE', #48809, #32526, #58819, .T. ) ;
#51337=DIRECTION ( 'NONE',  ( 0.000000000000000000, 0.000000000000000000, 1.000000000000000000 ) ) ;
#51338=VERTEX_POINT ( 'NONE', #3759 ) ;
#51340=DIRECTION ( 'NONE',  ( 0.000000000000000000, 1.000000000000000000, 0.000000000000000000 ) ) ;
#51341=DIRECTION ( 'NONE',  ( 0.000000000000000000, 1.000000000000000000, 0.000000000000000000 ) ) ;
#51342=ADVANCED_FACE ( 'NONE', ( #110488 ), #111107, .T. ) ;
#51343=EDGE_CURVE ( 'NONE', #107840, #2581, #6, .T. ) ;
#51344=EDGE_CURVE ( 'NONE', #79361, #46788, #127467, .T. ) ;
#51345=CONICAL_SURFACE ( 'NONE', #32565, 0.1000000000000000472, 0.003490658503988666988 ) ;
#51346=ORIENTED_EDGE ( 'NONE', *, *, #15812, .T. ) ;
#51347=DIRECTION ( 'NONE',  ( -0.000000000000000000, -1.000000000000000000, -0.000000000000000000 ) ) ;
#51348=ORIENTED_EDGE ( 'NONE', *, *, #118583, .F. ) ;
#51349=ORIENTED_EDGE ( 'NONE', *, *, #12863, .F. ) ;
#51350=CARTESIAN_POINT ( 'NONE',  ( -4.150000000000025224, 2.500000000000000000, -1.372243186433550033 ) ) ;
#51351=AXIS2_PLACEMENT_3D ( 'NONE', #125114, #35456, #3404 ) ;
#51352=ORIENTED_EDGE ( 'NONE', *, *, #52989, .F. ) ;
#51353=CARTESIAN_POINT ( 'NONE',  ( 18.27284318114482176, -0.4998542452738461428, -4.791717918554368794 ) ) ;
#51354=DIRECTION ( 'NONE',  ( 0.000000000000000000, -0.000000000000000000, 1.000000000000000000 ) ) ;
#51355=AXIS2_PLACEMENT_3D ( 'NONE', #38866, #98376, #78775 ) ;
#51356=AXIS2_PLACEMENT_3D ( 'NONE', #44924, #75646, #126704 ) ;
#51357=EDGE_LOOP ( 'NONE', ( #69064, #47897, #52759, #116116 ) ) ;
#51358=CARTESIAN_POINT ( 'NONE',  ( -3.950000000000026379, 12.50000000000000000, 6.776507416713035248 ) ) ;
#51359=DIRECTION ( 'NONE',  ( 0.000000000000000000, 1.000000000000000000, 0.000000000000000000 ) ) ;
#51360=ORIENTED_EDGE ( 'NONE', *, *, #30183, .F. ) ;
#51361=AXIS2_PLACEMENT_3D ( 'NONE', #43157, #92887, #12997 ) ;
#51362=ORIENTED_EDGE ( 'NONE', *, *, #33728, .F. ) ;
#51363=CONICAL_SURFACE ( 'NONE', #72201, 0.1000000000000002554, 0.003490658503988666988 ) ;
#51364=EDGE_LOOP ( 'NONE', ( #3371, #29749 ) ) ;
#51365=FACE_OUTER_BOUND ( 'NONE', #76716, .T. ) ;
#51366=FACE_OUTER_BOUND ( 'NONE', #13518, .T. ) ;
#51367=FACE_OUTER_BOUND ( 'NONE', #15308, .T. ) ;
#51368=FACE_BOUND ( 'NONE', #66000, .T. ) ;
#51369=EDGE_LOOP ( 'NONE', ( #27426, #63485, #71605, #105847 ) ) ;
#51370=DIRECTION ( 'NONE',  ( -4.274815082592931898E-19, -0.9999939076577903929, -0.003490651415223739937 ) ) ;
#51371=DIRECTION ( 'NONE',  ( -0.000000000000000000, 1.000000000000000000, -0.000000000000000000 ) ) ;
#51372=VERTEX_POINT ( 'NONE', #41130 ) ;
#51373=CARTESIAN_POINT ( 'NONE',  ( -6.650000000000014566, 12.50000000000000000, 5.802370205355744659 ) ) ;
#51374=AXIS2_PLACEMENT_3D ( 'NONE', #22558, #101748, #13989 ) ;
#51375=DIRECTION ( 'NONE',  ( -0.000000000000000000, -1.000000000000000000, -0.000000000000000000 ) ) ;
#51376=AXIS2_PLACEMENT_3D ( 'NONE', #128527, #89212, #28370 ) ;
#51377=CARTESIAN_POINT ( 'NONE',  ( -1.700000000000035261, 12.50000000000000000, 4.265033745738159077 ) ) ;
#51378=ADVANCED_FACE ( 'NONE', ( #10981 ), #12906, .T. ) ;
#51379=CARTESIAN_POINT ( 'NONE',  ( 1.049999999999953637, 12.50000000000000000, 2.511473670974873507 ) ) ;
#51380=CARTESIAN_POINT ( 'NONE',  ( -2.100000000000033396, 12.50000000000000000, -3.637306695894650055 ) ) ;
#51381=EDGE_CURVE ( 'NONE', #7787, #98954, #31340, .T. ) ;
#51382=CARTESIAN_POINT ( 'NONE',  ( -13.34999999999999076, 12.50000000000000000, -2.857883832488651521 ) ) ;
#51383=DIRECTION ( 'NONE',  ( 0.000000000000000000, 0.000000000000000000, -1.000000000000000000 ) ) ;
#51384=ADVANCED_FACE ( 'NONE', ( #3124 ), #66992, .T. ) ;
#51385=ORIENTED_EDGE ( 'NONE', *, *, #103171, .T. ) ;
#51386=VERTEX_POINT ( 'NONE', #120949 ) ;
#51387=EDGE_CURVE ( 'NONE', #128844, #41725, #46090, .T. ) ;
#51388=VERTEX_POINT ( 'NONE', #23385 ) ;
#51389=ORIENTED_EDGE ( 'NONE', *, *, #85160, .F. ) ;
#51390=DIRECTION ( 'NONE',  ( -0.000000000000000000, 1.000000000000000000, -0.000000000000000000 ) ) ;
#51391=ADVANCED_FACE ( 'NONE', ( #62050 ), #29374, .T. ) ;
#51392=CARTESIAN_POINT ( 'NONE',  ( 0.8499999999999557909, 12.50000000000000000, -7.253104124594891289 ) ) ;
#51393=ORIENTED_EDGE ( 'NONE', *, *, #92546, .F. ) ;
#51394=FACE_BOUND ( 'NONE', #31104, .T. ) ;
#51395=PLANE ( 'NONE',  #14421 ) ;
#51396=DIRECTION ( 'NONE',  ( 0.000000000000000000, 1.000000000000000000, 0.000000000000000000 ) ) ;
#51397=ADVANCED_FACE ( 'NONE', ( #100654 ), #35628, .T. ) ;
#51398=CARTESIAN_POINT ( 'NONE',  ( 4.149999999999941735, 2.500000000000000000, -1.372243186433550033 ) ) ;
#51399=ADVANCED_FACE ( 'NONE', ( #71206 ), #2161, .T. ) ;
#51400=VECTOR ( 'NONE', #57829, 1000.000000000000000 ) ;
#51401=DIRECTION ( 'NONE',  ( 0.000000000000000000, -0.000000000000000000, 1.000000000000000000 ) ) ;
#51402=AXIS2_PLACEMENT_3D ( 'NONE', #91867, #42121, #92497 ) ;
#51403=DIRECTION ( 'NONE',  ( 0.000000000000000000, 1.000000000000000000, 0.000000000000000000 ) ) ;
#51404=DIRECTION ( 'NONE',  ( 0.000000000000000000, -0.9999939076577903929, 0.003490651415223739937 ) ) ;
#51405=DIRECTION ( 'NONE',  ( -0.000000000000000000, -1.000000000000000000, -0.000000000000000000 ) ) ;
#51406=DIRECTION ( 'NONE',  ( 0.000000000000000000, -0.000000000000000000, 1.000000000000000000 ) ) ;
#51407=APPLICATION_CONTEXT ( 'automotive_design' ) ;
#51408=CARTESIAN_POINT ( 'NONE',  ( 11.89999999999990798, 2.500000000000000000, -4.776537180435977525 ) ) ;
#51409=EDGE_LOOP ( 'NONE', ( #56226, #91514 ) ) ;
#51410=ADVANCED_FACE ( 'NONE', ( #22778 ), #98298, .T. ) ;
#51411=EDGE_LOOP ( 'NONE', ( #118947, #8464, #71974, #43446 ) ) ;
#51412=EDGE_LOOP ( 'NONE', ( #97554, #81847 ) ) ;
#51413=ORIENTED_EDGE ( 'NONE', *, *, #49282, .T. ) ;
#51414=ORIENTED_EDGE ( 'NONE', *, *, #26378, .F. ) ;
#51415=ORIENTED_EDGE ( 'NONE', *, *, #35160, .F. ) ;
#51416=AXIS2_PLACEMENT_3D ( 'NONE', #29119, #100419, #49405 ) ;
#51418=VERTEX_POINT ( 'NONE', #62694 ) ;
#51419=VECTOR ( 'NONE', #117191, 1000.000000000000000 ) ;
#51420=AXIS2_PLACEMENT_3D ( 'NONE', #29523, #28886, #69431 ) ;
#51421=CARTESIAN_POINT ( 'NONE',  ( -3.950000000000029932, 2.500000000000000000, -6.048780366869526581 ) ) ;
#51422=CARTESIAN_POINT ( 'NONE',  ( -4.350000000000023626, 2.500000000000000000, -2.611473670974877592 ) ) ;
#51423=CARTESIAN_POINT ( 'NONE',  ( 10.64999999999990976, 2.500000000000000000, 1.918653347947321564 ) ) ;
#51424=CARTESIAN_POINT ( 'NONE',  ( -6.050000000000020250, 12.50000000000000000, -2.576566944158915184 ) ) ;
#51425=CONICAL_SURFACE ( 'NONE', #38618, 0.09999999999999999167, 0.003490658503988666988 ) ;
#51426=ORIENTED_EDGE ( 'NONE', *, *, #26387, .T. ) ;
#51427=DIRECTION ( 'NONE',  ( 0.000000000000000000, 0.000000000000000000, 1.000000000000000000 ) ) ;
#51428=ORIENTED_EDGE ( 'NONE', *, *, #13810, .T. ) ;
#51429=ORIENTED_EDGE ( 'NONE', *, *, #77646, .T. ) ;
#51430=CARTESIAN_POINT ( 'NONE',  ( 5.449999999999937117, 2.500000000000000000, -6.595190528383302109 ) ) ;
#51431=CARTESIAN_POINT ( 'NONE',  ( 5.599999999999934808, 2.500000000000000000, -4.676537180435978769 ) ) ;
#51432=FACE_OUTER_BOUND ( 'NONE', #58138, .T. ) ;
#51433=VECTOR ( 'NONE', #3883, 1000.000000000000000 ) ;
#51434=VERTEX_POINT ( 'NONE', #1814 ) ;
#51435=EDGE_LOOP ( 'NONE', ( #102547, #58406 ) ) ;
#51436=LINE ( 'NONE', #100507, #88132 ) ;
#51437=EDGE_CURVE ( 'NONE', #90278, #33163, #108762, .T. ) ;
#51438=CARTESIAN_POINT ( 'NONE',  ( -0.4500000000000402012, 2.500000000000000000, 2.065063509461097624 ) ) ;
#51439=DIRECTION ( 'NONE',  ( 0.000000000000000000, 0.000000000000000000, 1.000000000000000000 ) ) ;
#51440=CARTESIAN_POINT ( 'NONE',  ( -10.65000000000000391, 2.500000000000000000, -6.048780366869523029 ) ) ;
#51441=EDGE_LOOP ( 'NONE', ( #73891, #725 ) ) ;
#51442=DIRECTION ( 'NONE',  ( 0.000000000000000000, 0.000000000000000000, 1.000000000000000000 ) ) ;
#51443=CONICAL_SURFACE ( 'NONE', #30520, 0.09999999999999982514, 0.003490658503988666988 ) ;
#51444=ORIENTED_EDGE ( 'NONE', *, *, #126738, .F. ) ;
#51445=DIRECTION ( 'NONE',  ( 0.000000000000000000, -0.9999939076577903929, 0.003490651415223739937 ) ) ;
#51446=AXIS2_PLACEMENT_3D ( 'NONE', #31098, #33030, #100459 ) ;
#51447=ORIENTED_EDGE ( 'NONE', *, *, #22942, .F. ) ;
#51448=VECTOR ( 'NONE', #70672, 1000.000000000000000 ) ;
#51449=DIRECTION ( 'NONE',  ( -0.000000000000000000, -1.000000000000000000, -0.000000000000000000 ) ) ;
#51450=DIRECTION ( 'NONE',  ( -0.000000000000000000, -1.000000000000000000, -0.000000000000000000 ) ) ;
#51451=DIRECTION ( 'NONE',  ( 0.000000000000000000, 0.000000000000000000, 1.000000000000000000 ) ) ;
#51452=PLANE ( 'NONE',  #129591 ) ;
#51453=ORIENTED_EDGE ( 'NONE', *, *, #55468, .T. ) ;
#51454=CIRCLE ( 'NONE', #89096, 0.06509327318403745899 ) ;
#51455=CARTESIAN_POINT ( 'NONE',  ( 9.349999999999916156, 2.500000000000000000, 6.841600689897072485 ) ) ;
#51456=DIRECTION ( 'NONE',  ( 0.000000000000000000, -0.000000000000000000, 1.000000000000000000 ) ) ;
#51457=ORIENTED_EDGE ( 'NONE', *, *, #49201, .T. ) ;
#51458=VERTEX_POINT ( 'NONE', #43074 ) ;
#51460=DIRECTION ( 'NONE',  ( 0.000000000000000000, -0.000000000000000000, 1.000000000000000000 ) ) ;
#51461=FACE_OUTER_BOUND ( 'NONE', #51646, .T. ) ;
#51463=LINE ( 'NONE', #3632, #86696 ) ;
#51464=CARTESIAN_POINT ( 'NONE',  ( -5.850000000000019185, 2.500000000000000000, 6.495190528383297135 ) ) ;
#51465=CARTESIAN_POINT ( 'NONE',  ( -2.050000000000032685, 2.500000000000000000, -2.065063509461102065 ) ) ;
#51466=DIRECTION ( 'NONE',  ( 0.000000000000000000, -0.000000000000000000, 1.000000000000000000 ) ) ;
#51467=CARTESIAN_POINT ( 'NONE',  ( 2.049999999999950084, 2.500000000000000000, 2.265063509461097357 ) ) ;
#51468=EDGE_CURVE ( 'NONE', #88843, #17565, #77386, .T. ) ;
#51469=ORIENTED_EDGE ( 'NONE', *, *, #9097, .T. ) ;
#51470=DIRECTION ( 'NONE',  ( 0.000000000000000000, 0.000000000000000000, 1.000000000000000000 ) ) ;
#51472=CARTESIAN_POINT ( 'NONE',  ( 0.6499999999999561684, 12.50000000000000000, -2.576566944158915184 ) ) ;
#51473=DIRECTION ( 'NONE',  ( -4.274815082592931898E-19, -0.9999939076577903929, -0.003490651415223739937 ) ) ;
#51474=LINE ( 'NONE', #121476, #116981 ) ;
#51475=ADVANCED_FACE ( 'NONE', ( #122899 ), #125496, .T. ) ;
#51476=VERTEX_POINT ( 'NONE', #25990 ) ;
#51477=DIRECTION ( 'NONE',  ( -0.000000000000000000, -1.000000000000000000, -0.000000000000000000 ) ) ;
#51478=AXIS2_PLACEMENT_3D ( 'NONE', #37403, #129023, #66833 ) ;
#51479=AXIS2_PLACEMENT_3D ( 'NONE', #87821, #38100, #79329 ) ;
#51480=CARTESIAN_POINT ( 'NONE',  ( 1.249999999999988898, 2.500000000000000000, -6.595190528383302109 ) ) ;
#51481=LINE ( 'NONE', #3019, #100689 ) ;
#51482=ORIENTED_EDGE ( 'NONE', *, *, #100387, .F. ) ;
#51483=ADVANCED_FACE ( 'NONE', ( #14207 ), #83736, .T. ) ;
#51484=ADVANCED_FACE ( 'NONE', ( #46252 ), #12621, .T. ) ;
#51485=EDGE_CURVE ( 'NONE', #18602, #95183, #126106, .T. ) ;
#51486=ADVANCED_FACE ( 'NONE', ( #86159 ), #14669, .T. ) ;
#51487=EDGE_CURVE ( 'NONE', #9001, #40822, #20945, .T. ) ;
#51488=ORIENTED_EDGE ( 'NONE', *, *, #103124, .T. ) ;
#51489=CONICAL_SURFACE ( 'NONE', #70534, 0.1000000000000002554, 0.003490658503988666988 ) ;
#51490=DIRECTION ( 'NONE',  ( 0.000000000000000000, 0.000000000000000000, -1.000000000000000000 ) ) ;
#51491=ORIENTED_EDGE ( 'NONE', *, *, #117516, .F. ) ;
#51492=ORIENTED_EDGE ( 'NONE', *, *, #37970, .F. ) ;
#51493=CARTESIAN_POINT ( 'NONE',  ( -4.800000000000028244, 2.500000000000000000, -3.983716857408426293 ) ) ;
#51494=ADVANCED_FACE ( 'NONE', ( #46922 ), #75080, .T. ) ;
#51495=CARTESIAN_POINT ( 'NONE',  ( 21.23528140090977345, 2.699413673072324826, -2.293764360948901793 ) ) ;
#51496=CARTESIAN_POINT ( 'NONE',  ( 6.049999999999932321, 2.500000000000000000, 6.741600689897071952 ) ) ;
#51498=DIRECTION ( 'NONE',  ( 0.000000000000000000, 0.000000000000000000, -1.000000000000000000 ) ) ;
#51499=EDGE_LOOP ( 'NONE', ( #18229, #95582 ) ) ;
#51500=CONICAL_SURFACE ( 'NONE', #128883, 0.1000000000000000472, 0.003490658503988666988 ) ;
#51501=DIRECTION ( 'NONE',  ( 0.000000000000000000, 1.000000000000000000, 0.000000000000000000 ) ) ;
#51502=ORIENTED_EDGE ( 'NONE', *, *, #73831, .T. ) ;
#51503=DIRECTION ( 'NONE',  ( 0.000000000000000000, 0.000000000000000000, 1.000000000000000000 ) ) ;
#51504=DIRECTION ( 'NONE',  ( 0.000000000000000000, 0.000000000000000000, -1.000000000000000000 ) ) ;
#51505=ORIENTED_EDGE ( 'NONE', *, *, #44526, .T. ) ;
#51506=VERTEX_POINT ( 'NONE', #126766 ) ;
#51507=EDGE_LOOP ( 'NONE', ( #40348, #14000, #43841, #53100 ) ) ;
#51508=ORIENTED_EDGE ( 'NONE', *, *, #20910, .T. ) ;
#51509=DIRECTION ( 'NONE',  ( 0.000000000000000000, 1.000000000000000000, 0.000000000000000000 ) ) ;
#51510=CARTESIAN_POINT ( 'NONE',  ( 13.51931942407928311, 1.499999999999935829, 8.074217333073997693 ) ) ;
#51511=DIRECTION ( 'NONE',  ( 0.000000000000000000, 1.000000000000000000, 0.000000000000000000 ) ) ;
#51512=FACE_BOUND ( 'NONE', #26485, .T. ) ;
#51513=DIRECTION ( 'NONE',  ( 0.000000000000000000, 1.000000000000000000, 0.000000000000000000 ) ) ;
#51514=CIRCLE ( 'NONE', #11786, 0.1000000000000002554 ) ;
#51516=DIRECTION ( 'NONE',  ( 0.000000000000000000, 0.000000000000000000, 1.000000000000000000 ) ) ;
#51517=CARTESIAN_POINT ( 'NONE',  ( -10.85000000000000142, 2.500000000000000000, -6.495190528383298911 ) ) ;
#51518=VECTOR ( 'NONE', #29758, 1000.000000000000000 ) ;
#51519=AXIS2_PLACEMENT_3D ( 'NONE', #44178, #84098, #84760 ) ;
#51520=DIRECTION ( 'NONE',  ( 0.000000000000000000, 1.000000000000000000, 0.000000000000000000 ) ) ;
#51521=CIRCLE ( 'NONE', #91226, 0.06509327318403745899 ) ;
#51522=DIRECTION ( 'NONE',  ( -4.274815082592931898E-19, -0.9999939076577903929, -0.003490651415223739937 ) ) ;
#51523=EDGE_CURVE ( 'NONE', #75902, #121648, #56698, .T. ) ;
#51524=DIRECTION ( 'NONE',  ( 0.000000000000000000, -0.9999939076577903929, 0.003490651415223739937 ) ) ;
#51525=AXIS2_PLACEMENT_3D ( 'NONE', #121870, #23672, #121227 ) ;
#51526=EDGE_CURVE ( 'NONE', #73897, #123363, #104570, .T. ) ;
#51527=VECTOR ( 'NONE', #102862, 1000.000000000000000 ) ;
#51528=DIRECTION ( 'NONE',  ( -0.000000000000000000, 1.000000000000000000, -0.000000000000000000 ) ) ;
#51529=CIRCLE ( 'NONE', #124686, 0.06509327318403741736 ) ;
#51530=EDGE_CURVE ( 'NONE', #74881, #55968, #96008, .T. ) ;
#51531=ORIENTED_EDGE ( 'NONE', *, *, #70989, .F. ) ;
#51532=ORIENTED_EDGE ( 'NONE', *, *, #5367, .T. ) ;
#51533=ORIENTED_EDGE ( 'NONE', *, *, #100146, .T. ) ;
#51534=VERTEX_POINT ( 'NONE', #103898 ) ;
#51535=VERTEX_POINT ( 'NONE', #63974 ) ;
#51536=DIRECTION ( 'NONE',  ( 0.000000000000000000, 1.000000000000000000, 0.000000000000000000 ) ) ;
#51537=DIRECTION ( 'NONE',  ( -0.000000000000000000, 1.000000000000000000, -0.000000000000000000 ) ) ;
#51538=ORIENTED_EDGE ( 'NONE', *, *, #127638, .T. ) ;
#51539=EDGE_CURVE ( 'NONE', #84566, #34168, #55438, .T. ) ;
#51540=FACE_BOUND ( 'NONE', #92029, .T. ) ;
#51541=CARTESIAN_POINT ( 'NONE',  ( 1.449999999999949551, 2.500000000000000000, 6.841600689897072485 ) ) ;
#51542=EDGE_CURVE ( 'NONE', #20680, #78871, #94712, .T. ) ;
#51543=ADVANCED_FACE ( 'NONE', ( #124180 ), #33576, .T. ) ;
#51544=CIRCLE ( 'NONE', #3410, 0.06509327318403745899 ) ;
#51545=VECTOR ( 'NONE', #100172, 1000.000000000000000 ) ;
#51546=EDGE_CURVE ( 'NONE', #121027, #56893, #43942, .T. ) ;
#51547=ORIENTED_EDGE ( 'NONE', *, *, #13287, .F. ) ;
#51548=DIRECTION ( 'NONE',  ( -0.000000000000000000, -1.000000000000000000, -0.000000000000000000 ) ) ;
#51549=CARTESIAN_POINT ( 'NONE',  ( 3.549999999999943867, 12.50000000000000000, -6.148780366869526226 ) ) ;
#51550=DIRECTION ( 'NONE',  ( 0.000000000000000000, 0.000000000000000000, 1.000000000000000000 ) ) ;
#51551=DIRECTION ( 'NONE',  ( 0.000000000000000000, -0.9999939076577903929, 0.003490651415223739937 ) ) ;
#51552=ORIENTED_EDGE ( 'NONE', *, *, #79411, .F. ) ;
#51553=LINE ( 'NONE', #60720, #88910 ) ;
#51554=ADVANCED_FACE ( 'NONE', ( #65239 ), #79536, .T. ) ;
#51555=VERTEX_POINT ( 'NONE', #5672 ) ;
#51556=ORIENTED_EDGE ( 'NONE', *, *, #103403, .F. ) ;
#51557=DIRECTION ( 'NONE',  ( 0.000000000000000000, 0.000000000000000000, 1.000000000000000000 ) ) ;
#51558=DIRECTION ( 'NONE',  ( 0.000000000000000000, 0.000000000000000000, -1.000000000000000000 ) ) ;
#51559=ORIENTED_EDGE ( 'NONE', *, *, #15268, .F. ) ;
#51560=DIRECTION ( 'NONE',  ( -0.000000000000000000, -1.000000000000000000, -0.000000000000000000 ) ) ;
#51561=CARTESIAN_POINT ( 'NONE',  ( 11.89999999999990798, 2.500000000000000000, 3.883716857408421319 ) ) ;
#51562=LINE ( 'NONE', #120927, #72878 ) ;
#51563=DIRECTION ( 'NONE',  ( 0.000000000000000000, -0.000000000000000000, 1.000000000000000000 ) ) ;
#51565=ORIENTED_EDGE ( 'NONE', *, *, #44535, .T. ) ;
#51566=DIRECTION ( 'NONE',  ( 0.000000000000000000, 1.000000000000000000, 0.000000000000000000 ) ) ;
#51567=ADVANCED_FACE ( 'NONE', ( #54780 ), #127560, .T. ) ;
#51568=EDGE_LOOP ( 'NONE', ( #48622, #111255, #99443, #25629 ) ) ;
#51569=FACE_OUTER_BOUND ( 'NONE', #99958, .T. ) ;
#51570=AXIS2_PLACEMENT_3D ( 'NONE', #107415, #110635, #120459 ) ;
#51571=EDGE_LOOP ( 'NONE', ( #3419, #66894, #121269, #109351 ) ) ;
#51572=FACE_OUTER_BOUND ( 'NONE', #5728, .T. ) ;
#51573=VERTEX_POINT ( 'NONE', #6309 ) ;
#51574=CARTESIAN_POINT ( 'NONE',  ( 1.049999999999953637, 12.50000000000000000, 2.576566944158910744 ) ) ;
#51575=CARTESIAN_POINT ( 'NONE',  ( -10.40000000000000213, 12.50000000000000000, -0.7579135962115916003 ) ) ;
#51576=DIRECTION ( 'NONE',  ( 0.000000000000000000, 0.000000000000000000, 1.000000000000000000 ) ) ;
#51577=PLANE ( 'NONE',  #660 ) ;
#51578=CARTESIAN_POINT ( 'NONE',  ( 16.89731025888663041, 0.9183091266721068457, -5.698390440797600931 ) ) ;
#51579=ORIENTED_EDGE ( 'NONE', *, *, #113001, .T. ) ;
#51580=VECTOR ( 'NONE', #3341, 1000.000000000000000 ) ;
#51581=AXIS2_PLACEMENT_3D ( 'NONE', #73088, #123463, #34470 ) ;
#51582=ORIENTED_EDGE ( 'NONE', *, *, #100856, .T. ) ;
#51583=ORIENTED_EDGE ( 'NONE', *, *, #94770, .T. ) ;
#51584=DIRECTION ( 'NONE',  ( 0.000000000000000000, 1.000000000000000000, 0.000000000000000000 ) ) ;
#51585=ADVANCED_FACE ( 'NONE', ( #26623 ), #96235, .T. ) ;
#51586=PLANE ( 'NONE',  #7604 ) ;
#51587=DIRECTION ( 'NONE',  ( 0.000000000000000000, 0.000000000000000000, -1.000000000000000000 ) ) ;
#51588=VERTEX_POINT ( 'NONE', #115633 ) ;
#51589=ORIENTED_EDGE ( 'NONE', *, *, #110864, .T. ) ;
#51590=EDGE_LOOP ( 'NONE', ( #60480, #127476, #76073, #33282 ) ) ;
#51591=DIRECTION ( 'NONE',  ( -0.000000000000000000, 1.000000000000000000, -0.000000000000000000 ) ) ;
#51592=CONICAL_SURFACE ( 'NONE', #59919, 0.1000000000000002554, 0.003490658503988666988 ) ;
#51593=AXIS2_PLACEMENT_3D ( 'NONE', #98187, #8503, #76626 ) ;
#51594=ORIENTED_EDGE ( 'NONE', *, *, #13783, .T. ) ;
#51595=PLANE ( 'NONE',  #128124 ) ;
#51596=DIRECTION ( 'NONE',  ( -0.000000000000000000, -1.000000000000000000, -0.000000000000000000 ) ) ;
#51597=AXIS2_PLACEMENT_3D ( 'NONE', #66058, #66699, #57541 ) ;
#51598=DIRECTION ( 'NONE',  ( -0.000000000000000000, 1.000000000000000000, -0.000000000000000000 ) ) ;
#51599=CARTESIAN_POINT ( 'NONE',  ( -10.00000000000000355, 12.50000000000000000, 3.702399969078682407 ) ) ;
#51600=DIRECTION ( 'NONE',  ( 0.000000000000000000, 0.000000000000000000, -1.000000000000000000 ) ) ;
#51601=DIRECTION ( 'NONE',  ( -0.000000000000000000, 1.000000000000000000, -0.000000000000000000 ) ) ;
#51602=CARTESIAN_POINT ( 'NONE',  ( -3.550000000000027356, 12.50000000000000000, 1.818653347947321475 ) ) ;
#51603=EDGE_CURVE ( 'NONE', #114390, #126294, #23101, .T. ) ;
#51604=CARTESIAN_POINT ( 'NONE',  ( 10.84999999999991260, 12.50000000000000000, 7.188010851410848723 ) ) ;
#51605=ORIENTED_EDGE ( 'NONE', *, *, #5063, .T. ) ;
#51606=CARTESIAN_POINT ( 'NONE',  ( -0.6500000000000394351, 2.500000000000000000, 2.511473670974873507 ) ) ;
#51607=CARTESIAN_POINT ( 'NONE',  ( 59.74180401148688446, -3.401974578037520125, 5.439313020096691709 ) ) ;
#51608=EDGE_LOOP ( 'NONE', ( #3275, #121431 ) ) ;
#51609=ORIENTED_EDGE ( 'NONE', *, *, #92994, .T. ) ;
#51611=CARTESIAN_POINT ( 'NONE',  ( 0.6499999999999561684, 2.500000000000000000, -2.611473670974877592 ) ) ;
#51612=DIRECTION ( 'NONE',  ( 0.000000000000000000, 1.000000000000000000, 0.000000000000000000 ) ) ;
#51613=CARTESIAN_POINT ( 'NONE',  ( -1.450000000000035483, 12.50000000000000000, 1.818653347947321475 ) ) ;
#51614=DIRECTION ( 'NONE',  ( 0.000000000000000000, 1.000000000000000000, 0.000000000000000000 ) ) ;
#51615=DIRECTION ( 'NONE',  ( 0.000000000000000000, 0.000000000000000000, -1.000000000000000000 ) ) ;
#51616=VECTOR ( 'NONE', #125861, 1000.000000000000000 ) ;
#51617=FACE_OUTER_BOUND ( 'NONE', #11022, .T. ) ;
#51618=CARTESIAN_POINT ( 'NONE',  ( -12.04999999999999716, 2.500000000000000000, -2.165063509461097713 ) ) ;
#51619=CIRCLE ( 'NONE', #53662, 0.06509327318403745899 ) ;
#51620=CIRCLE ( 'NONE', #39115, 0.06509327318403745899 ) ;
#51621=CARTESIAN_POINT ( 'NONE',  ( -10.20000000000000462, 12.50000000000000000, 4.676537180435972552 ) ) ;
#51622=EDGE_LOOP ( 'NONE', ( #18241, #87619 ) ) ;
#51623=ORIENTED_EDGE ( 'NONE', *, *, #68368, .T. ) ;
#51624=AXIS2_PLACEMENT_3D ( 'NONE', #115193, #74019, #84483 ) ;
#51625=EDGE_CURVE ( 'NONE', #5536, #42483, #73265, .T. ) ;
#51626=ORIENTED_EDGE ( 'NONE', *, *, #101498, .F. ) ;
#51627=ORIENTED_EDGE ( 'NONE', *, *, #23877, .F. ) ;
#51628=AXIS2_PLACEMENT_3D ( 'NONE', #104048, #24842, #66688 ) ;
#51629=DIRECTION ( 'NONE',  ( -0.000000000000000000, 1.000000000000000000, -0.000000000000000000 ) ) ;
#51630=CARTESIAN_POINT ( 'NONE',  ( -4.800000000000022915, 12.50000000000000000, 3.983716857408420076 ) ) ;
#51631=AXIS2_PLACEMENT_3D ( 'NONE', #83857, #44591, #23018 ) ;
#51632=EDGE_LOOP ( 'NONE', ( #65107, #40244 ) ) ;
#51633=CARTESIAN_POINT ( 'NONE',  ( -3.150000000000029221, 12.50000000000000000, 2.511473670974873507 ) ) ;
#51634=CARTESIAN_POINT ( 'NONE',  ( -4.150000000000024336, 12.50000000000000000, 1.537336459617582918 ) ) ;
#51635=AXIS2_PLACEMENT_3D ( 'NONE', #3605, #12123, #83473 ) ;
#51636=AXIS2_PLACEMENT_3D ( 'NONE', #46385, #106601, #104036 ) ;
#51638=CARTESIAN_POINT ( 'NONE',  ( 14.14999999999989200, 2.500000000000000000, -2.165063509461101710 ) ) ;
#51639=ORIENTED_EDGE ( 'NONE', *, *, #12762, .T. ) ;
#51640=EDGE_CURVE ( 'NONE', #9353, #7114, #89982, .T. ) ;
#51641=ADVANCED_FACE ( 'NONE', ( #8898 ), #77639, .T. ) ;
#51642=ADVANCED_FACE ( 'NONE', ( #69771 ), #100546, .T. ) ;
#51643=CARTESIAN_POINT ( 'NONE',  ( -4.999999999999990230, 2.500000000000000000, -4.430127018922202176 ) ) ;
#51644=EDGE_CURVE ( 'NONE', #74427, #86526, #21036, .T. ) ;
#51646=EDGE_LOOP ( 'NONE', ( #63033, #13854, #23332, #129315 ) ) ;
#51647=EDGE_CURVE ( 'NONE', #26349, #77466, #27254, .T. ) ;
#51648=EDGE_LOOP ( 'NONE', ( #55986, #1439 ) ) ;
#51649=ORIENTED_EDGE ( 'NONE', *, *, #76014, .F. ) ;
#51650=ORIENTED_EDGE ( 'NONE', *, *, #73083, .F. ) ;
#51651=CARTESIAN_POINT ( 'NONE',  ( 11.64999999999990621, 2.500000000000000000, 6.395190528383296602 ) ) ;
#51652=AXIS2_PLACEMENT_3D ( 'NONE', #67812, #88071, #18713 ) ;
#51653=EDGE_CURVE ( 'NONE', #93502, #126749, #98388, .T. ) ;
#51654=DIRECTION ( 'NONE',  ( 0.000000000000000000, 0.000000000000000000, 1.000000000000000000 ) ) ;
#51655=LINE ( 'NONE', #22200, #115149 ) ;
#51656=EDGE_CURVE ( 'NONE', #32318, #118375, #112883, .T. ) ;
#51657=EDGE_CURVE ( 'NONE', #24428, #87918, #4279, .T. ) ;
#51658=ORIENTED_EDGE ( 'NONE', *, *, #48269, .F. ) ;
#51659=LINE ( 'NONE', #100104, #100417 ) ;
#51660=ORIENTED_EDGE ( 'NONE', *, *, #57775, .F. ) ;
#51661=DIRECTION ( 'NONE',  ( 0.000000000000000000, -0.000000000000000000, 1.000000000000000000 ) ) ;
#51662=DIRECTION ( 'NONE',  ( 0.000000000000000000, -0.000000000000000000, 1.000000000000000000 ) ) ;
#51663=CARTESIAN_POINT ( 'NONE',  ( -3.300000000000027800, 2.500000000000000000, 0.09999999999999772959 ) ) ;
#51664=CARTESIAN_POINT ( 'NONE',  ( 0.3999999999999559464, 12.50000000000000000, -4.265033745738164406 ) ) ;
#51665=EDGE_CURVE ( 'NONE', #122222, #12736, #127644, .T. ) ;
#51666=EDGE_LOOP ( 'NONE', ( #41652, #17343, #26195, #59676 ) ) ;
#51667=VECTOR ( 'NONE', #7112, 1000.000000000000000 ) ;
#51668=AXIS2_PLACEMENT_3D ( 'NONE', #20568, #69007, #100415 ) ;
#51669=ORIENTED_EDGE ( 'NONE', *, *, #60954, .F. ) ;
#51670=VERTEX_POINT ( 'NONE', #97295 ) ;
#51671=CARTESIAN_POINT ( 'NONE',  ( 5.649999999999936406, 2.500000000000000000, -6.941600689897077459 ) ) ;
#51672=DIRECTION ( 'NONE',  ( 0.000000000000000000, 0.000000000000000000, 1.000000000000000000 ) ) ;
#51673=FACE_BOUND ( 'NONE', #109802, .T. ) ;
#51674=DIRECTION ( 'NONE',  ( 0.000000000000000000, 0.000000000000000000, 1.000000000000000000 ) ) ;
#51675=LINE ( 'NONE', #11732, #80045 ) ;
#51676=AXIS2_PLACEMENT_3D ( 'NONE', #2499, #32001, #43759 ) ;
#51677=DIRECTION ( 'NONE',  ( -0.000000000000000000, -1.000000000000000000, -0.000000000000000000 ) ) ;
#51678=CARTESIAN_POINT ( 'NONE',  ( 10.84999999999990905, 12.50000000000000000, -5.802370205355749988 ) ) ;
#51680=DIRECTION ( 'NONE',  ( 0.000000000000000000, -0.9999939076577903929, 0.003490651415223739937 ) ) ;
#51681=EDGE_LOOP ( 'NONE', ( #77081, #15868 ) ) ;
#51682=VECTOR ( 'NONE', #109061, 1000.000000000000000 ) ;
#51683=VECTOR ( 'NONE', #76475, 1000.000000000000000 ) ;
#51684=DIRECTION ( 'NONE',  ( -0.000000000000000000, 1.000000000000000000, -0.000000000000000000 ) ) ;
#51685=AXIS2_PLACEMENT_3D ( 'NONE', #81479, #101113, #91291 ) ;
#51686=FACE_OUTER_BOUND ( 'NONE', #59228, .T. ) ;
#51687=VERTEX_POINT ( 'NONE', #88768 ) ;
#51688=ORIENTED_EDGE ( 'NONE', *, *, #64332, .F. ) ;
#51689=CARTESIAN_POINT ( 'NONE',  ( -11.44999999999999751, 12.50000000000000000, 2.576566944158910744 ) ) ;
#51690=DIRECTION ( 'NONE',  ( 0.000000000000000000, 0.000000000000000000, 1.000000000000000000 ) ) ;
#51691=FACE_BOUND ( 'NONE', #20793, .T. ) ;
#51692=LINE ( 'NONE', #98835, #5441 ) ;
#51693=EDGE_CURVE ( 'NONE', #30477, #29851, #7614, .T. ) ;
#51694=EDGE_CURVE ( 'NONE', #12100, #53692, #56610, .T. ) ;
#51695=ORIENTED_EDGE ( 'NONE', *, *, #19844, .T. ) ;
#51696=DIRECTION ( 'NONE',  ( 0.000000000000000000, 0.000000000000000000, -1.000000000000000000 ) ) ;
#51698=ORIENTED_EDGE ( 'NONE', *, *, #61890, .T. ) ;
#51699=FACE_OUTER_BOUND ( 'NONE', #118946, .T. ) ;
#51700=CARTESIAN_POINT ( 'NONE',  ( 9.799999999999915445, 12.50000000000000000, 3.983716857408420964 ) ) ;
#51701=EDGE_CURVE ( 'NONE', #100575, #43976, #77472, .T. ) ;
#51702=CIRCLE ( 'NONE', #16069, 0.1000000000000000056 ) ;
#51703=CARTESIAN_POINT ( 'NONE',  ( -14.59999999999998366, 2.500000000000000000, 0.09999999999999989453 ) ) ;
#51704=DIRECTION ( 'NONE',  ( -0.000000000000000000, -1.000000000000000000, -0.000000000000000000 ) ) ;
#51705=AXIS2_PLACEMENT_3D ( 'NONE', #84702, #122696, #122063 ) ;
#51706=AXIS2_PLACEMENT_3D ( 'NONE', #22739, #14165, #113681 ) ;
#51707=ORIENTED_EDGE ( 'NONE', *, *, #117578, .F. ) ;
#51708=VECTOR ( 'NONE', #123083, 1000.000000000000000 ) ;
#51709=VECTOR ( 'NONE', #116507, 1000.000000000000000 ) ;
#51710=DIRECTION ( 'NONE',  ( 0.000000000000000000, 1.000000000000000000, 0.000000000000000000 ) ) ;
#51711=CARTESIAN_POINT ( 'NONE',  ( -0.8500000000000390576, 12.50000000000000000, -6.495190528383302464 ) ) ;
#51712=FACE_OUTER_BOUND ( 'NONE', #71107, .T. ) ;
#51713=ORIENTED_EDGE ( 'NONE', *, *, #23708, .T. ) ;
#51714=ORIENTED_EDGE ( 'NONE', *, *, #54126, .F. ) ;
#51715=CONICAL_SURFACE ( 'NONE', #110206, 0.1000000000000000472, 0.003490658503988666988 ) ;
#51716=CARTESIAN_POINT ( 'NONE',  ( -6.650000000000018119, 2.500000000000000000, -2.757883832488654097 ) ) ;
#51717=ORIENTED_EDGE ( 'NONE', *, *, #119905, .T. ) ;
#51718=CARTESIAN_POINT ( 'NONE',  ( 0.4499999999999569344, 2.500000000000000000, -2.165063509461101710 ) ) ;
#51719=FACE_OUTER_BOUND ( 'NONE', #76573, .T. ) ;
#51720=CIRCLE ( 'NONE', #116452, 0.06509327318403745899 ) ;
#51721=AXIS2_PLACEMENT_3D ( 'NONE', #56995, #100627, #10942 ) ;
#51722=DIRECTION ( 'NONE',  ( -4.274815082592931898E-19, -0.9999939076577903929, -0.003490651415223739937 ) ) ;
#51723=ORIENTED_EDGE ( 'NONE', *, *, #101021, .F. ) ;
#51724=DIRECTION ( 'NONE',  ( -0.000000000000000000, -1.000000000000000000, -0.000000000000000000 ) ) ;
#51725=DIRECTION ( 'NONE',  ( -0.000000000000000000, 1.000000000000000000, -0.000000000000000000 ) ) ;
#51726=DIRECTION ( 'NONE',  ( -0.000000000000000000, 1.000000000000000000, -0.000000000000000000 ) ) ;
#51727=( BOUNDED_SURFACE ( )  B_SPLINE_SURFACE ( 3, 2, ( 
 ( #14167, #63938, #44283 ),
 ( #26591, #67793, #100957 ),
 ( #36427, #126725, #8225 ),
 ( #127373, #70223, #17386 ) ),
 .UNSPECIFIED., .F., .F., .F. ) 
 B_SPLINE_SURFACE_WITH_KNOTS ( ( 4, 4 ),
 ( 3, 3 ),
 ( -9.367506770274758310E-17, 0.002140783067917591091 ),
 ( 0.000000000000000000, 1.000000000000000000 ),
 .UNSPECIFIED. ) 
 GEOMETRIC_REPRESENTATION_ITEM ( )  RATIONAL_B_SPLINE_SURFACE ( (
 ( 1.000000000000000000, 0.7071067811865473507, 1.000000000000000000),
 ( 1.000000000000000000, 0.7083221562484182110, 1.000000000000000000),
 ( 1.000000000000000000, 0.7095583416414843470, 1.000000000000000000),
 ( 1.000000000000000000, 0.7108129113927461606, 1.000000000000000000) ) ) 
 REPRESENTATION_ITEM ( '' )  SURFACE ( )  );
#51728=FACE_OUTER_BOUND ( 'NONE', #81477, .T. ) ;
#51730=CARTESIAN_POINT ( 'NONE',  ( -12.69999999999999218, 2.500000000000000000, -0.3464101615137741286 ) ) ;
#51731=ORIENTED_EDGE ( 'NONE', *, *, #97197, .T. ) ;
#51732=ORIENTED_EDGE ( 'NONE', *, *, #87990, .T. ) ;
#51733=CARTESIAN_POINT ( 'NONE',  ( 4.999999999999973355, 12.50000000000000000, -4.330127018922201643 ) ) ;
#51734=ORIENTED_EDGE ( 'NONE', *, *, #119756, .F. ) ;
#51736=VERTEX_POINT ( 'NONE', #97936 ) ;
#51737=EDGE_LOOP ( 'NONE', ( #66316, #30079 ) ) ;
#51738=ORIENTED_EDGE ( 'NONE', *, *, #123563, .T. ) ;
#51739=AXIS2_PLACEMENT_3D ( 'NONE', #4491, #64090, #96123 ) ;
#51740=CARTESIAN_POINT ( 'NONE',  ( 11.84999999999990727, 2.500000000000000000, -2.611473670974877592 ) ) ;
#51741=PLANE ( 'NONE',  #65308 ) ;
#51742=DIRECTION ( 'NONE',  ( -0.000000000000000000, -1.000000000000000000, -0.000000000000000000 ) ) ;
#51743=CARTESIAN_POINT ( 'NONE',  ( -0.8500000000000395017, 12.50000000000000000, 2.099970236277060032 ) ) ;
#51744=PLANE ( 'NONE',  #64703 ) ;
#51746=EDGE_CURVE ( 'NONE', #45239, #36155, #31507, .T. ) ;
#51747=LINE ( 'NONE', #53034, #76892 ) ;
#51748=LINE ( 'NONE', #83775, #57077 ) ;
#51749=EDGE_CURVE ( 'NONE', #128241, #49718, #125574, .T. ) ;
#51750=CARTESIAN_POINT ( 'NONE',  ( -2.950000000000029932, 12.50000000000000000, 2.165063509461097713 ) ) ;
#51751=CIRCLE ( 'NONE', #124904, 0.1000000000000002554 ) ;
#51752=VERTEX_POINT ( 'NONE', #29219 ) ;
#51753=AXIS2_PLACEMENT_3D ( 'NONE', #36839, #14588, #95749 ) ;
#51754=DIRECTION ( 'NONE',  ( 0.000000000000000000, -0.000000000000000000, 1.000000000000000000 ) ) ;
#51755=ORIENTED_EDGE ( 'NONE', *, *, #22245, .T. ) ;
#51757=EDGE_LOOP ( 'NONE', ( #38936, #29240, #23828, #69924 ) ) ;
#51758=CARTESIAN_POINT ( 'NONE',  ( -11.25000000000000000, 12.50000000000000000, 2.922977105672686982 ) ) ;
#51759=CARTESIAN_POINT ( 'NONE',  ( 9.999999999999948486, 2.500000000000000000, 4.430127018922196847 ) ) ;
#51760=CARTESIAN_POINT ( 'NONE',  ( 10.84999999999990905, 2.500000000000000000, 2.857883832488649301 ) ) ;
#51761=CONICAL_SURFACE ( 'NONE', #80999, 0.1000000000000002554, 0.003490658503988666988 ) ;
#51762=AXIS2_PLACEMENT_3D ( 'NONE', #91551, #71926, #41826 ) ;
#51763=CARTESIAN_POINT ( 'NONE',  ( 4.149999999999939959, 12.50000000000000000, -2.230156782645139391 ) ) ;
#51764=CIRCLE ( 'NONE', #106132, 0.1000000000000002554 ) ;
#51765=CARTESIAN_POINT ( 'NONE',  ( -12.89999999999999147, 2.500000000000000000, 4.330127018922196314 ) ) ;
#51766=CARTESIAN_POINT ( 'NONE',  ( 5.199999999999935341, 12.50000000000000000, -3.983716857408426293 ) ) ;
#51767=CARTESIAN_POINT ( 'NONE',  ( 10.84999999999991260, 12.50000000000000000, -2.857883832488653741 ) ) ;
#51768=VERTEX_POINT ( 'NONE', #9565 ) ;
#51769=VERTEX_POINT ( 'NONE', #49507 ) ;
#51770=AXIS2_PLACEMENT_3D ( 'NONE', #21760, #110763, #40109 ) ;
#51771=ORIENTED_EDGE ( 'NONE', *, *, #37048, .T. ) ;
#51772=EDGE_CURVE ( 'NONE', #121109, #97069, #104645, .T. ) ;
#51773=ORIENTED_EDGE ( 'NONE', *, *, #41958, .T. ) ;
#51774=ORIENTED_EDGE ( 'NONE', *, *, #48276, .T. ) ;
#51775=DIRECTION ( 'NONE',  ( 0.000000000000000000, 0.000000000000000000, -1.000000000000000000 ) ) ;
#51776=CARTESIAN_POINT ( 'NONE',  ( 2.899999999999945732, 2.500000000000000000, -2.385244779468109755E-15 ) ) ;
#51777=ADVANCED_FACE ( 'NONE', ( #12760 ), #73352, .T. ) ;
#51778=AXIS2_PLACEMENT_3D ( 'NONE', #80849, #73581, #44795 ) ;
#51779=DIRECTION ( 'NONE',  ( 0.000000000000000000, 0.000000000000000000, 1.000000000000000000 ) ) ;
#51780=CARTESIAN_POINT ( 'NONE',  ( -10.84999999999999964, 2.500000000000000000, 5.902370205355745192 ) ) ;
#51781=AXIS2_PLACEMENT_3D ( 'NONE', #83452, #1639, #91968 ) ;
#51782=DIRECTION ( 'NONE',  ( -0.000000000000000000, -1.000000000000000000, -0.000000000000000000 ) ) ;
#51783=ORIENTED_EDGE ( 'NONE', *, *, #83564, .F. ) ;
#51784=CARTESIAN_POINT ( 'NONE',  ( -6.700000000000019718, 2.500000000000000000, -2.385244779468109755E-15 ) ) ;
#51785=DIRECTION ( 'NONE',  ( 0.000000000000000000, 0.000000000000000000, 1.000000000000000000 ) ) ;
#51786=EDGE_CURVE ( 'NONE', #53209, #74697, #72994, .T. ) ;
#51787=EDGE_CURVE ( 'NONE', #18239, #61946, #58698, .T. ) ;
#51788=CARTESIAN_POINT ( 'NONE',  ( -13.29999999999998828, 2.500000000000000000, 4.330127018922196314 ) ) ;
#51789=ADVANCED_FACE ( 'NONE', ( #40325 ), #117246, .T. ) ;
#51790=DIRECTION ( 'NONE',  ( 0.000000000000000000, 0.000000000000000000, 1.000000000000000000 ) ) ;
#51791=CIRCLE ( 'NONE', #124937, 0.1000000000000002554 ) ;
#51792=EDGE_CURVE ( 'NONE', #84812, #3294, #103094, .T. ) ;
#51793=DIRECTION ( 'NONE',  ( 0.000000000000000000, 0.000000000000000000, -1.000000000000000000 ) ) ;
#51794=ORIENTED_EDGE ( 'NONE', *, *, #58726, .T. ) ;
#51795=CIRCLE ( 'NONE', #118581, 0.09999999999999999167 ) ;
#51796=VERTEX_POINT ( 'NONE', #112285 ) ;
#51797=EDGE_CURVE ( 'NONE', #53658, #25872, #62543, .T. ) ;
#51798=VERTEX_POINT ( 'NONE', #70416 ) ;
#51799=DIRECTION ( 'NONE',  ( 0.000000000000000000, 1.000000000000000000, 0.000000000000000000 ) ) ;
#51800=ADVANCED_FACE ( 'NONE', ( #82829 ), #30516, .T. ) ;
#51801=CIRCLE ( 'NONE', #93651, 0.06509327318403745899 ) ;
#51802=ORIENTED_EDGE ( 'NONE', *, *, #89115, .F. ) ;
#51803=CIRCLE ( 'NONE', #3668, 0.1000000000000002554 ) ;
#51804=DIRECTION ( 'NONE',  ( 0.000000000000000000, -0.9999939076577903929, 0.003490651415223739937 ) ) ;
#51806=EDGE_CURVE ( 'NONE', #121634, #67054, #71062, .T. ) ;
#51807=CONICAL_SURFACE ( 'NONE', #101976, 0.1000000000000000472, 0.003490658503988666988 ) ;
#51808=EDGE_CURVE ( 'NONE', #75922, #25044, #75409, .T. ) ;
#51810=DIRECTION ( 'NONE',  ( 0.000000000000000000, 0.000000000000000000, 1.000000000000000000 ) ) ;
#51811=CARTESIAN_POINT ( 'NONE',  ( 12.49999999999990408, 2.500000000000000000, 5.122947341949749323 ) ) ;
#51812=CIRCLE ( 'NONE', #124959, 0.1000000000000002554 ) ;
#51813=DIRECTION ( 'NONE',  ( 0.000000000000000000, 0.000000000000000000, 1.000000000000000000 ) ) ;
#51814=PLANE ( 'NONE',  #129320 ) ;
#51815=ADVANCED_FACE ( 'NONE', ( #122737 ), #12700, .T. ) ;
#51816=AXIS2_PLACEMENT_3D ( 'NONE', #23747, #24385, #13903 ) ;
#51817=CIRCLE ( 'NONE', #118700, 0.1000000000000002554 ) ;
#51818=DIRECTION ( 'NONE',  ( 0.000000000000000000, 0.000000000000000000, 1.000000000000000000 ) ) ;
#51819=VERTEX_POINT ( 'NONE', #12125 ) ;
#51820=ORIENTED_EDGE ( 'NONE', *, *, #26758, .F. ) ;
#51821=FACE_OUTER_BOUND ( 'NONE', #71666, .T. ) ;
#51822=CARTESIAN_POINT ( 'NONE',  ( -4.800000000000022915, 2.500000000000000000, -0.2464101615137783419 ) ) ;
#51823=DIRECTION ( 'NONE',  ( 0.000000000000000000, 0.000000000000000000, -1.000000000000000000 ) ) ;
#51824=FACE_OUTER_BOUND ( 'NONE', #47416, .T. ) ;
#51825=EDGE_LOOP ( 'NONE', ( #14871, #83628 ) ) ;
#51826=ORIENTED_EDGE ( 'NONE', *, *, #110301, .F. ) ;
#51827=CARTESIAN_POINT ( 'NONE',  ( -0.6000000000000383915, 2.500000000000000000, -3.883716857408426648 ) ) ;
#51828=DIRECTION ( 'NONE',  ( 0.000000000000000000, -0.000000000000000000, 1.000000000000000000 ) ) ;
#51829=DIRECTION ( 'NONE',  ( 0.000000000000000000, -0.000000000000000000, 1.000000000000000000 ) ) ;
#51830=LINE ( 'NONE', #33487, #36318 ) ;
#51831=EDGE_LOOP ( 'NONE', ( #52184, #103908 ) ) ;
#51832=DIRECTION ( 'NONE',  ( 0.000000000000000000, -0.000000000000000000, 1.000000000000000000 ) ) ;
#51833=CARTESIAN_POINT ( 'NONE',  ( -1.650000000000034772, 12.50000000000000000, 1.472243186433545459 ) ) ;
#51834=VERTEX_POINT ( 'NONE', #52076 ) ;
#51835=CIRCLE ( 'NONE', #20541, 0.06509327318403745899 ) ;
#51836=DIRECTION ( 'NONE',  ( 0.000000000000000000, 0.000000000000000000, -1.000000000000000000 ) ) ;
#51837=EDGE_LOOP ( 'NONE', ( #127075, #57780 ) ) ;
#51838=DIRECTION ( 'NONE',  ( -0.000000000000000000, -1.000000000000000000, -0.000000000000000000 ) ) ;
#51839=AXIS2_PLACEMENT_3D ( 'NONE', #96968, #29530, #89094 ) ;
#51840=ORIENTED_EDGE ( 'NONE', *, *, #40519, .F. ) ;
#51841=ADVANCED_FACE ( 'NONE', ( #91986 ), #81675, .T. ) ;
#51842=AXIS2_PLACEMENT_3D ( 'NONE', #97675, #38119, #47299 ) ;
#51843=EDGE_LOOP ( 'NONE', ( #6197, #98843 ) ) ;
#51844=DIRECTION ( 'NONE',  ( -4.274815082592931898E-19, -0.9999939076577903929, -0.003490651415223739937 ) ) ;
#51845=CARTESIAN_POINT ( 'NONE',  ( 9.599999999999914380, 2.500000000000000000, -5.022947341949754119 ) ) ;
#51846=EDGE_CURVE ( 'NONE', #87255, #124518, #64942, .T. ) ;
#51847=ORIENTED_EDGE ( 'NONE', *, *, #84264, .F. ) ;
#51848=EDGE_LOOP ( 'NONE', ( #84859, #80965 ) ) ;
#51849=FACE_OUTER_BOUND ( 'NONE', #52911, .T. ) ;
#51850=CARTESIAN_POINT ( 'NONE',  ( -1.250000000000037526, 12.50000000000000000, -1.472243186433550122 ) ) ;
#51851=AXIS2_PLACEMENT_3D ( 'NONE', #112612, #109550, #113236 ) ;
#51854=AXIS2_PLACEMENT_3D ( 'NONE', #20904, #2534, #71953 ) ;
#51855=PLANE ( 'NONE',  #114347 ) ;
#51856=CARTESIAN_POINT ( 'NONE',  ( -12.09999999999999609, 2.500000000000000000, -0.09999999999999827083 ) ) ;
#51857=CARTESIAN_POINT ( 'NONE',  ( 3.349999999999943689, 2.500000000000000000, 2.065063509461097624 ) ) ;
#51858=DIRECTION ( 'NONE',  ( -4.274815082592931898E-19, -0.9999939076577903929, -0.003490651415223739937 ) ) ;
#51859=DIRECTION ( 'NONE',  ( -4.274815082592931898E-19, -0.9999939076577903929, -0.003490651415223739937 ) ) ;
#51860=AXIS2_PLACEMENT_3D ( 'NONE', #87741, #116561, #108033 ) ;
#51861=VERTEX_POINT ( 'NONE', #120164 ) ;
#51862=ORIENTED_EDGE ( 'NONE', *, *, #67390, .T. ) ;
#51863=DIRECTION ( 'NONE',  ( 0.000000000000000000, 0.000000000000000000, 1.000000000000000000 ) ) ;
#51864=ORIENTED_EDGE ( 'NONE', *, *, #68158, .T. ) ;
#51865=DIRECTION ( 'NONE',  ( 0.000000000000000000, 1.000000000000000000, 0.000000000000000000 ) ) ;
#51866=DIRECTION ( 'NONE',  ( 0.000000000000000000, 0.000000000000000000, -1.000000000000000000 ) ) ;
#51867=AXIS2_PLACEMENT_3D ( 'NONE', #63044, #70931, #51313 ) ;
#51868=CARTESIAN_POINT ( 'NONE',  ( -5.650000000000019895, 2.500000000000000000, 6.148780366869520009 ) ) ;
#51869=ORIENTED_EDGE ( 'NONE', *, *, #39649, .F. ) ;
#51870=ORIENTED_EDGE ( 'NONE', *, *, #74124, .T. ) ;
#51871=FACE_BOUND ( 'NONE', #106285, .T. ) ;
#51872=ORIENTED_EDGE ( 'NONE', *, *, #58291, .F. ) ;
#51873=CARTESIAN_POINT ( 'NONE',  ( 14.14999999999989555, 2.500000000000000000, 2.165063509461097713 ) ) ;
#51874=CARTESIAN_POINT ( 'NONE',  ( 1.049999999999954081, 2.500000000000000000, -6.148780366869526226 ) ) ;
#51875=DIRECTION ( 'NONE',  ( 0.000000000000000000, 0.000000000000000000, -1.000000000000000000 ) ) ;
#51876=CONICAL_SURFACE ( 'NONE', #125020, 0.1000000000000002554, 0.003490658503988666988 ) ;
#51877=CARTESIAN_POINT ( 'NONE',  ( 8.749999999999953815, 12.50000000000000000, -2.165063509461101710 ) ) ;
#51878=FACE_OUTER_BOUND ( 'NONE', #63722, .T. ) ;
#51879=CARTESIAN_POINT ( 'NONE',  ( -3.350000000000028955, 2.500000000000000000, -2.165063509461101710 ) ) ;
#51880=CONICAL_SURFACE ( 'NONE', #125023, 0.1000000000000002554, 0.003490658503988666988 ) ;
#51881=FACE_OUTER_BOUND ( 'NONE', #2132, .T. ) ;
#51883=CARTESIAN_POINT ( 'NONE',  ( 9.199999999999915801, 12.50000000000000000, -4.330127018922201643 ) ) ;
#51884=FACE_OUTER_BOUND ( 'NONE', #117492, .T. ) ;
#51885=AXIS2_PLACEMENT_3D ( 'NONE', #196, #92453, #13886 ) ;
#51886=CIRCLE ( 'NONE', #68590, 0.1000000000000002554 ) ;
#51887=FACE_OUTER_BOUND ( 'NONE', #55791, .T. ) ;
#51888=EDGE_CURVE ( 'NONE', #60383, #75351, #20679, .T. ) ;
#51889=ORIENTED_EDGE ( 'NONE', *, *, #96751, .F. ) ;
#51891=VERTEX_POINT ( 'NONE', #50778 ) ;
#51892=ORIENTED_EDGE ( 'NONE', *, *, #80299, .F. ) ;
#51893=CARTESIAN_POINT ( 'NONE',  ( -0.8500000000000395017, 12.50000000000000000, 2.165063509461097713 ) ) ;
#51894=ORIENTED_EDGE ( 'NONE', *, *, #73769, .T. ) ;
#51895=CARTESIAN_POINT ( 'NONE',  ( 7.049999999999930544, 2.500000000000000000, -6.595190528383302109 ) ) ;
#51896=CARTESIAN_POINT ( 'NONE',  ( 7.699999999999925571, 2.500000000000000000, 4.083716857408420609 ) ) ;
#51897=ORIENTED_EDGE ( 'NONE', *, *, #111689, .F. ) ;
#51898=ORIENTED_EDGE ( 'NONE', *, *, #78394, .F. ) ;
#51899=AXIS2_PLACEMENT_3D ( 'NONE', #4047, #42724, #104190 ) ;
#51900=ORIENTED_EDGE ( 'NONE', *, *, #124039, .F. ) ;
#51901=PLANE ( 'NONE',  #8296 ) ;
#51902=DIRECTION ( 'NONE',  ( 0.000000000000000000, -0.000000000000000000, 1.000000000000000000 ) ) ;
#51903=DIRECTION ( 'NONE',  ( 0.000000000000000000, 0.000000000000000000, -1.000000000000000000 ) ) ;
#51904=LINE ( 'NONE', #99067, #91019 ) ;
#51905=CARTESIAN_POINT ( 'NONE',  ( -2.100000000000034284, 2.500000000000000000, -2.385244779468109755E-15 ) ) ;
#51906=EDGE_CURVE ( 'NONE', #98420, #28344, #90701, .T. ) ;
#51907=FACE_OUTER_BOUND ( 'NONE', #111615, .T. ) ;
#51908=ADVANCED_FACE ( 'NONE', ( #72362 ), #80891, .T. ) ;
#51909=ORIENTED_EDGE ( 'NONE', *, *, #13087, .F. ) ;
#51911=VERTEX_POINT ( 'NONE', #31156 ) ;
#51912=VECTOR ( 'NONE', #74776, 1000.000000000000000 ) ;
#51913=VECTOR ( 'NONE', #78709, 1000.000000000000000 ) ;
#51914=VERTEX_POINT ( 'NONE', #1662 ) ;
#51915=ORIENTED_EDGE ( 'NONE', *, *, #16450, .T. ) ;
#51916=FACE_OUTER_BOUND ( 'NONE', #100706, .T. ) ;
#51917=VERTEX_POINT ( 'NONE', #110962 ) ;
#51918=ADVANCED_FACE ( 'NONE', ( #21304 ), #117153, .T. ) ;
#51919=VERTEX_POINT ( 'NONE', #105680 ) ;
#51920=ORIENTED_EDGE ( 'NONE', *, *, #105281, .F. ) ;
#51923=DIRECTION ( 'NONE',  ( 0.000000000000000000, 1.000000000000000000, 0.000000000000000000 ) ) ;
#51924=LINE ( 'NONE', #62389, #77728 ) ;
#51925=DIRECTION ( 'NONE',  ( -0.000000000000000000, -1.000000000000000000, -0.000000000000000000 ) ) ;
#51926=FACE_OUTER_BOUND ( 'NONE', #45803, .T. ) ;
#51927=AXIS2_PLACEMENT_3D ( 'NONE', #109471, #59752, #12543 ) ;
#51928=DIRECTION ( 'NONE',  ( -0.000000000000000000, 1.000000000000000000, -0.000000000000000000 ) ) ;
#51929=ORIENTED_EDGE ( 'NONE', *, *, #19368, .F. ) ;
#51930=AXIS2_PLACEMENT_3D ( 'NONE', #53712, #13778, #73344 ) ;
#51931=DIRECTION ( 'NONE',  ( -4.274815082592931898E-19, -0.9999939076577903929, -0.003490651415223739937 ) ) ;
#51932=EDGE_LOOP ( 'NONE', ( #61507, #32056, #26556, #93126 ) ) ;
#51933=DIRECTION ( 'NONE',  ( 0.000000000000000000, 0.000000000000000000, -1.000000000000000000 ) ) ;
#51934=AXIS2_PLACEMENT_3D ( 'NONE', #41909, #121732, #84393 ) ;
#51935=ORIENTED_EDGE ( 'NONE', *, *, #15312, .T. ) ;
#51936=CARTESIAN_POINT ( 'NONE',  ( -7.100000000000013856, 2.500000000000000000, 5.022947341949748790 ) ) ;
#51937=ORIENTED_EDGE ( 'NONE', *, *, #15615, .F. ) ;
#51938=CIRCLE ( 'NONE', #54071, 0.1000000000000002554 ) ;
#51941=EDGE_CURVE ( 'NONE', #99488, #97111, #75556, .T. ) ;
#51942=LINE ( 'NONE', #91860, #71870 ) ;
#51943=ORIENTED_EDGE ( 'NONE', *, *, #38862, .F. ) ;
#51944=ORIENTED_EDGE ( 'NONE', *, *, #116787, .F. ) ;
#51945=DIRECTION ( 'NONE',  ( -0.000000000000000000, -1.000000000000000000, -0.000000000000000000 ) ) ;
#51946=FACE_OUTER_BOUND ( 'NONE', #121510, .T. ) ;
#51947=ADVANCED_FACE ( 'NONE', ( #24537 ), #102597, .T. ) ;
#51948=DIRECTION ( 'NONE',  ( -4.274815082592931898E-19, -0.9999939076577903929, -0.003490651415223739937 ) ) ;
#51949=DIRECTION ( 'NONE',  ( 0.000000000000000000, -0.9999939076577903929, 0.003490651415223739937 ) ) ;
#51950=VECTOR ( 'NONE', #39138, 1000.000000000000000 ) ;
#51951=ADVANCED_FACE ( 'NONE', ( #66389 ), #62901, .T. ) ;
#51952=FACE_OUTER_BOUND ( 'NONE', #80534, .T. ) ;
#51953=CIRCLE ( 'NONE', #127258, 0.09999999999999999167 ) ;
#51954=ORIENTED_EDGE ( 'NONE', *, *, #34948, .F. ) ;
#51955=CARTESIAN_POINT ( 'NONE',  ( 7.499999999999927169, 2.500000000000000000, 3.737306695894644371 ) ) ;
#51957=EDGE_CURVE ( 'NONE', #77408, #27361, #15984, .T. ) ;
#51958=EDGE_CURVE ( 'NONE', #4494, #69514, #42071, .T. ) ;
#51959=ADVANCED_FACE ( 'NONE', ( #5520 ), #98471, .T. ) ;
#51960=ORIENTED_EDGE ( 'NONE', *, *, #24741, .F. ) ;
#51961=DIRECTION ( 'NONE',  ( 0.000000000000000000, -0.000000000000000000, 1.000000000000000000 ) ) ;
#51962=FACE_OUTER_BOUND ( 'NONE', #52965, .T. ) ;
#51963=AXIS2_PLACEMENT_3D ( 'NONE', #7744, #77764, #117680 ) ;
#51964=EDGE_CURVE ( 'NONE', #97550, #34514, #29545, .T. ) ;
#51965=DIRECTION ( 'NONE',  ( 0.000000000000000000, 0.000000000000000000, -1.000000000000000000 ) ) ;
#51966=CARTESIAN_POINT ( 'NONE',  ( 10.84999999999990905, 2.500000000000000000, 1.472243186433545459 ) ) ;
#51967=DIRECTION ( 'NONE',  ( -4.274815082592931898E-19, -0.9999939076577903929, -0.003490651415223739937 ) ) ;
#51969=CARTESIAN_POINT ( 'NONE',  ( 0.5999999999999551248, 12.50000000000000000, -4.611443907251940644 ) ) ;
#51970=ORIENTED_EDGE ( 'NONE', *, *, #68161, .F. ) ;
#51971=ADVANCED_FACE ( 'NONE', ( #74290 ), #92219, .T. ) ;
#51972=CONICAL_SURFACE ( 'NONE', #79069, 0.1000000000000002554, 0.003490658503988666988 ) ;
#51973=CARTESIAN_POINT ( 'NONE',  ( -5.400000000000023448, 2.500000000000000000, -4.330127018922201643 ) ) ;
#51974=DIRECTION ( 'NONE',  ( 0.000000000000000000, 0.000000000000000000, 1.000000000000000000 ) ) ;
#51975=CARTESIAN_POINT ( 'NONE',  ( 3.749999999999942268, 12.50000000000000000, -5.802370205355749988 ) ) ;
#51976=ORIENTED_EDGE ( 'NONE', *, *, #123535, .F. ) ;
#51977=ORIENTED_EDGE ( 'NONE', *, *, #50834, .F. ) ;
#51978=CONICAL_SURFACE ( 'NONE', #39387, 0.1000000000000002554, 0.003490658503988666988 ) ;
#51979=CARTESIAN_POINT ( 'NONE',  ( 9.349999999999916156, 12.50000000000000000, -2.446380397790840266 ) ) ;
#51980=AXIS2_PLACEMENT_3D ( 'NONE', #63564, #74660, #113948 ) ;
#51981=ORIENTED_EDGE ( 'NONE', *, *, #68294, .F. ) ;
#51982=EDGE_LOOP ( 'NONE', ( #92094, #108763, #109899, #127018 ) ) ;
#51983=DIRECTION ( 'NONE',  ( 0.000000000000000000, -0.9999939076577903929, 0.003490651415223739937 ) ) ;
#51984=EDGE_LOOP ( 'NONE', ( #51239, #15569 ) ) ;
#51985=DIRECTION ( 'NONE',  ( -0.000000000000000000, 1.000000000000000000, -0.000000000000000000 ) ) ;
#51986=CONICAL_SURFACE ( 'NONE', #129368, 0.1000000000000002554, 0.003490658503988666988 ) ;
#51987=DIRECTION ( 'NONE',  ( 0.000000000000000000, 0.000000000000000000, -1.000000000000000000 ) ) ;
#51988=CARTESIAN_POINT ( 'NONE',  ( 11.64999999999990798, 12.50000000000000000, 5.737276932171707422 ) ) ;
#51989=ORIENTED_EDGE ( 'NONE', *, *, #46038, .F. ) ;
#51990=CARTESIAN_POINT ( 'NONE',  ( 9.599999999999914380, 12.50000000000000000, 4.330127018922196314 ) ) ;
#51991=AXIS2_PLACEMENT_3D ( 'NONE', #117799, #18322, #58270 ) ;
#51992=FACE_OUTER_BOUND ( 'NONE', #15116, .T. ) ;
#51993=ORIENTED_EDGE ( 'NONE', *, *, #48516, .F. ) ;
#51994=CIRCLE ( 'NONE', #125153, 0.1000000000000000056 ) ;
#51995=AXIS2_PLACEMENT_3D ( 'NONE', #94785, #113790, #33933 ) ;
#51996=EDGE_CURVE ( 'NONE', #89246, #113013, #46256, .T. ) ;
#51997=EDGE_LOOP ( 'NONE', ( #122165, #81476, #28725, #93208 ) ) ;
#51998=ORIENTED_EDGE ( 'NONE', *, *, #31119, .T. ) ;
#51999=DIRECTION ( 'NONE',  ( -4.274815082592931898E-19, -0.9999939076577903929, -0.003490651415223739937 ) ) ;
#52000=FACE_OUTER_BOUND ( 'NONE', #1126, .T. ) ;
#52001=LINE ( 'NONE', #80817, #8744 ) ;
#52002=FACE_BOUND ( 'NONE', #107066, .T. ) ;
#52003=EDGE_LOOP ( 'NONE', ( #126311, #19170, #83675, #109104 ) ) ;
#52004=CARTESIAN_POINT ( 'NONE',  ( 10.19999999999991580, 12.50000000000000000, -0.4115034346978157509 ) ) ;
#52005=DIRECTION ( 'NONE',  ( 0.000000000000000000, 1.000000000000000000, 0.000000000000000000 ) ) ;
#52006=EDGE_LOOP ( 'NONE', ( #13827, #81416 ) ) ;
#52007=EDGE_CURVE ( 'NONE', #12189, #87317, #93924, .T. ) ;
#52008=CARTESIAN_POINT ( 'NONE',  ( -13.94999999999998863, 2.500000000000000000, 2.611473670974877148 ) ) ;
#52009=DIRECTION ( 'NONE',  ( -4.274815082592931898E-19, -0.9999939076577903929, -0.003490651415223739937 ) ) ;
#52010=CARTESIAN_POINT ( 'NONE',  ( 7.499999999999960032, 2.500000000000000000, -2.276824562219559311E-15 ) ) ;
#52011=FACE_OUTER_BOUND ( 'NONE', #13286, .T. ) ;
#52012=VECTOR ( 'NONE', #115087, 1000.000000000000000 ) ;
#52013=CARTESIAN_POINT ( 'NONE',  ( 1.649999999999950617, 12.50000000000000000, 2.165063509461097713 ) ) ;
#52014=DIRECTION ( 'NONE',  ( 0.000000000000000000, -0.9999939076577903929, 0.003490651415223739937 ) ) ;
#52015=DIRECTION ( 'NONE',  ( 0.000000000000000000, 1.000000000000000000, 0.000000000000000000 ) ) ;
#52016=VECTOR ( 'NONE', #81720, 1000.000000000000000 ) ;
#52017=AXIS2_PLACEMENT_3D ( 'NONE', #69630, #19898, #120027 ) ;
#52018=ORIENTED_EDGE ( 'NONE', *, *, #46641, .T. ) ;
#52019=ORIENTED_EDGE ( 'NONE', *, *, #48287, .T. ) ;
#52020=AXIS2_PLACEMENT_3D ( 'NONE', #105829, #123525, #85543 ) ;
#52021=ORIENTED_EDGE ( 'NONE', *, *, #118862, .F. ) ;
#52022=ORIENTED_EDGE ( 'NONE', *, *, #76603, .F. ) ;
#52023=CARTESIAN_POINT ( 'NONE',  ( 6.249999999999928946, 2.500000000000000000, 2.957883832488649389 ) ) ;
#52024=CARTESIAN_POINT ( 'NONE',  ( -2.700000000000030376, 12.50000000000000000, 3.983716857408420964 ) ) ;
#52025=ORIENTED_EDGE ( 'NONE', *, *, #86845, .F. ) ;
#52026=FACE_BOUND ( 'NONE', #1079, .T. ) ;
#52027=CARTESIAN_POINT ( 'NONE',  ( 6.249999999999932498, 12.50000000000000000, 5.802370205355744659 ) ) ;
#52028=DIRECTION ( 'NONE',  ( 0.000000000000000000, 1.000000000000000000, 0.000000000000000000 ) ) ;
#52029=AXIS2_PLACEMENT_3D ( 'NONE', #8768, #109576, #29099 ) ;
#52030=CIRCLE ( 'NONE', #97981, 0.06509327318403745899 ) ;
#52031=DIRECTION ( 'NONE',  ( -0.000000000000000000, -1.000000000000000000, -0.000000000000000000 ) ) ;
#52032=CIRCLE ( 'NONE', #118916, 0.1000000000000002554 ) ;
#52033=DIRECTION ( 'NONE',  ( 0.000000000000000000, 1.000000000000000000, 0.000000000000000000 ) ) ;
#52034=DIRECTION ( 'NONE',  ( 0.000000000000000000, 0.000000000000000000, 1.000000000000000000 ) ) ;
#52035=CARTESIAN_POINT ( 'NONE',  ( -6.050000000000017586, 2.500000000000000000, 6.048780366869520364 ) ) ;
#52036=LINE ( 'NONE', #42881, #20384 ) ;
#52037=DIRECTION ( 'NONE',  ( 0.000000000000000000, 0.000000000000000000, -1.000000000000000000 ) ) ;
#52038=DIRECTION ( 'NONE',  ( 0.000000000000000000, 0.000000000000000000, 1.000000000000000000 ) ) ;
#52039=AXIS2_PLACEMENT_3D ( 'NONE', #93360, #86087, #123449 ) ;
#52040=ORIENTED_EDGE ( 'NONE', *, *, #4789, .T. ) ;
#52041=CIRCLE ( 'NONE', #60466, 0.06509327318403745899 ) ;
#52042=ADVANCED_FACE ( 'NONE', ( #114209 ), #15337, .T. ) ;
#52043=ORIENTED_EDGE ( 'NONE', *, *, #88300, .F. ) ;
#52044=VERTEX_POINT ( 'NONE', #35027 ) ;
#52045=ORIENTED_EDGE ( 'NONE', *, *, #58926, .F. ) ;
#52046=ORIENTED_EDGE ( 'NONE', *, *, #96960, .T. ) ;
#52047=VERTEX_POINT ( 'NONE', #55290 ) ;
#52048=CARTESIAN_POINT ( 'NONE',  ( 7.499999999999925393, 12.50000000000000000, 5.022947341949748790 ) ) ;
#52049=ORIENTED_EDGE ( 'NONE', *, *, #74349, .F. ) ;
#52050=ORIENTED_EDGE ( 'NONE', *, *, #88238, .T. ) ;
#52051=CIRCLE ( 'NONE', #29073, 0.06509327318403743123 ) ;
#52052=EDGE_CURVE ( 'NONE', #59320, #73842, #6512, .T. ) ;
#52053=FACE_OUTER_BOUND ( 'NONE', #23070, .T. ) ;
#52054=CARTESIAN_POINT ( 'NONE',  ( 13.80679872452937396, -2.499999999999552802, 7.946844944429471980 ) ) ;
#52055=CARTESIAN_POINT ( 'NONE',  ( -1.250000000000037970, 2.500000000000000000, 2.857883832488649301 ) ) ;
#52056=DIRECTION ( 'NONE',  ( 0.000000000000000000, -0.000000000000000000, 1.000000000000000000 ) ) ;
#52057=CIRCLE ( 'NONE', #49913, 0.06509327318403745899 ) ;
#52058=EDGE_CURVE ( 'NONE', #23160, #98765, #127739, .T. ) ;
#52060=VERTEX_POINT ( 'NONE', #125314 ) ;
#52061=DIRECTION ( 'NONE',  ( 0.000000000000000000, 0.000000000000000000, -1.000000000000000000 ) ) ;
#52062=ORIENTED_EDGE ( 'NONE', *, *, #71907, .F. ) ;
#52064=AXIS2_PLACEMENT_3D ( 'NONE', #49522, #8919, #8281 ) ;
#52065=DIRECTION ( 'NONE',  ( 0.000000000000000000, 1.000000000000000000, 0.000000000000000000 ) ) ;
#52066=EDGE_CURVE ( 'NONE', #75250, #75194, #23267, .T. ) ;
#52067=DIRECTION ( 'NONE',  ( -0.000000000000000000, 1.000000000000000000, -0.000000000000000000 ) ) ;
#52068=EDGE_CURVE ( 'NONE', #65715, #38578, #119402, .T. ) ;
#52069=VERTEX_POINT ( 'NONE', #78161 ) ;
#52070=AXIS2_PLACEMENT_3D ( 'NONE', #59832, #48695, #119352 ) ;
#52071=ORIENTED_EDGE ( 'NONE', *, *, #75858, .F. ) ;
#52072=FACE_OUTER_BOUND ( 'NONE', #76029, .T. ) ;
#52073=AXIS2_PLACEMENT_3D ( 'NONE', #75941, #66765, #86401 ) ;
#52074=CARTESIAN_POINT ( 'NONE',  ( -13.29999999999998828, 2.500000000000000000, 4.430127018922196847 ) ) ;
#52075=DIRECTION ( 'NONE',  ( -0.000000000000000000, 1.000000000000000000, -0.000000000000000000 ) ) ;
#52076=CARTESIAN_POINT ( 'NONE',  ( -7.900000000000011013, 12.50000000000000000, 4.395220292106234439 ) ) ;
#52077=CARTESIAN_POINT ( 'NONE',  ( -4.600000000000024514, 2.500000000000000000, 3.637306695894644726 ) ) ;
#52078=ORIENTED_EDGE ( 'NONE', *, *, #49462, .F. ) ;
#52079=DIRECTION ( 'NONE',  ( 0.000000000000000000, -0.000000000000000000, 1.000000000000000000 ) ) ;
#52080=ORIENTED_EDGE ( 'NONE', *, *, #28024, .T. ) ;
#52081=CARTESIAN_POINT ( 'NONE',  ( 17.50000000000000000, 2.499999999999999556, -3.333333333333329485 ) ) ;
#52082=AXIS2_PLACEMENT_3D ( 'NONE', #97655, #7978, #78015 ) ;
#52083=CIRCLE ( 'NONE', #18618, 0.09999999999999982514 ) ;
#52084=CARTESIAN_POINT ( 'NONE',  ( -10.40000000000000391, 12.50000000000000000, -3.702399969078682851 ) ) ;
#52085=CARTESIAN_POINT ( 'NONE',  ( -7.900000000000014566, 2.500000000000000000, 0.5928203230275495006 ) ) ;
#52086=CIRCLE ( 'NONE', #39584, 0.06509327318403745899 ) ;
#52087=CARTESIAN_POINT ( 'NONE',  ( -10.60000000000000320, 12.50000000000000000, -3.918623584224384615 ) ) ;
#52088=DIRECTION ( 'NONE',  ( 0.000000000000000000, 0.000000000000000000, 1.000000000000000000 ) ) ;
#52089=VERTEX_POINT ( 'NONE', #117395 ) ;
#52090=FACE_OUTER_BOUND ( 'NONE', #67644, .T. ) ;
#52091=CONICAL_SURFACE ( 'NONE', #37430, 0.1000000000000000472, 0.003490658503988666988 ) ;
#52092=LINE ( 'NONE', #22640, #125944 ) ;
#52093=ORIENTED_EDGE ( 'NONE', *, *, #116162, .T. ) ;
#52094=ORIENTED_EDGE ( 'NONE', *, *, #117072, .T. ) ;
#52095=EDGE_LOOP ( 'NONE', ( #96240, #96387 ) ) ;
#52096=CARTESIAN_POINT ( 'NONE',  ( 2.500000000000002220, -2.750000000000000444, 10.00000000000000178 ) ) ;
#52097=DIRECTION ( 'NONE',  ( -0.000000000000000000, -1.000000000000000000, -0.000000000000000000 ) ) ;
#52098=CARTESIAN_POINT ( 'NONE',  ( 8.349999999999919709, 12.50000000000000000, -1.472243186433550122 ) ) ;
#52099=FACE_OUTER_BOUND ( 'NONE', #101032, .T. ) ;
#52100=EDGE_CURVE ( 'NONE', #15328, #30332, #35803, .T. ) ;
#52101=LINE ( 'NONE', #25198, #96984 ) ;
#52102=DIRECTION ( 'NONE',  ( 0.000000000000000000, 0.000000000000000000, 1.000000000000000000 ) ) ;
#52103=CARTESIAN_POINT ( 'NONE',  ( 5.199999999999933564, 2.500000000000000000, 0.4464101615137735513 ) ) ;
#52104=ADVANCED_FACE ( 'NONE', ( #119353 ), #126615, .T. ) ;
#52105=AXIS2_PLACEMENT_3D ( 'NONE', #42205, #9015, #48972 ) ;
#52106=EDGE_CURVE ( 'NONE', #31758, #115693, #28412, .T. ) ;
#52107=EDGE_CURVE ( 'NONE', #10471, #50344, #77550, .T. ) ;
#52108=EDGE_CURVE ( 'NONE', #126779, #89530, #8111, .T. ) ;
#52109=CIRCLE ( 'NONE', #106477, 0.09999999999999982514 ) ;
#52110=AXIS2_PLACEMENT_3D ( 'NONE', #29402, #98120, #28760 ) ;
#52112=ADVANCED_FACE ( 'NONE', ( #6792 ), #94280, .T. ) ;
#52113=CARTESIAN_POINT ( 'NONE',  ( 8.149999999999920419, 12.50000000000000000, -2.446380397790840266 ) ) ;
#52114=CARTESIAN_POINT ( 'NONE',  ( -9.350000000000004974, 12.50000000000000000, 6.148780366869520897 ) ) ;
#52115=DIRECTION ( 'NONE',  ( 0.000000000000000000, 1.000000000000000000, 0.000000000000000000 ) ) ;
#52116=DIRECTION ( 'NONE',  ( -0.000000000000000000, 1.000000000000000000, -0.000000000000000000 ) ) ;
#52117=ORIENTED_EDGE ( 'NONE', *, *, #122085, .F. ) ;
#52118=AXIS2_PLACEMENT_3D ( 'NONE', #37114, #58042, #48210 ) ;
#52119=ADVANCED_FACE ( 'NONE', ( #8740 ), #71293, .T. ) ;
#52120=CARTESIAN_POINT ( 'NONE',  ( -1.250000000000037970, 12.50000000000000000, 2.857883832488649301 ) ) ;
#52121=AXIS2_PLACEMENT_3D ( 'NONE', #96957, #87135, #115961 ) ;
#52122=EDGE_CURVE ( 'NONE', #97182, #104775, #16972, .T. ) ;
#52123=DIRECTION ( 'NONE',  ( -4.274815082592931898E-19, -0.9999939076577903929, -0.003490651415223739937 ) ) ;
#52124=DIRECTION ( 'NONE',  ( -0.000000000000000000, -1.000000000000000000, -0.000000000000000000 ) ) ;
#52125=VERTEX_POINT ( 'NONE', #109549 ) ;
#52126=AXIS2_PLACEMENT_3D ( 'NONE', #85307, #54544, #125244 ) ;
#52128=CARTESIAN_POINT ( 'NONE',  ( -13.09999999999999254, 2.500000000000000000, -0.3464101615137741286 ) ) ;
#52129=CONICAL_SURFACE ( 'NONE', #12400, 0.1000000000000002554, 0.003490658503988666988 ) ;
#52130=CIRCLE ( 'NONE', #31308, 0.06509327318403745899 ) ;
#52131=ORIENTED_EDGE ( 'NONE', *, *, #3242, .F. ) ;
#52132=ORIENTED_EDGE ( 'NONE', *, *, #80307, .F. ) ;
#52133=DIRECTION ( 'NONE',  ( 0.000000000000000000, 1.000000000000000000, 0.000000000000000000 ) ) ;
#52134=CARTESIAN_POINT ( 'NONE',  ( 20.80581321129326255, 0.6997403544423165256, -4.161084241360471836 ) ) ;
#52135=LINE ( 'NONE', #41041, #88143 ) ;
#52136=FACE_OUTER_BOUND ( 'NONE', #78608, .T. ) ;
#52137=ORIENTED_EDGE ( 'NONE', *, *, #28925, .F. ) ;
#52138=DIRECTION ( 'NONE',  ( 0.000000000000000000, 0.000000000000000000, 1.000000000000000000 ) ) ;
#52139=VERTEX_POINT ( 'NONE', #48697 ) ;
#52140=CONICAL_SURFACE ( 'NONE', #85579, 0.09999999999999982514, 0.003490658503988666988 ) ;
#52141=CARTESIAN_POINT ( 'NONE',  ( 17.49100792770887125, 2.144659849951620068, 4.220823783472687829 ) ) ;
#52143=EDGE_LOOP ( 'NONE', ( #104936, #120431 ) ) ;
#52144=ORIENTED_EDGE ( 'NONE', *, *, #24906, .F. ) ;
#52145=ORIENTED_EDGE ( 'NONE', *, *, #111580, .T. ) ;
#52146=EDGE_LOOP ( 'NONE', ( #42169, #26229, #93399, #85795 ) ) ;
#52147=CARTESIAN_POINT ( 'NONE',  ( 6.649999999999930189, 12.50000000000000000, -2.857883832488653741 ) ) ;
#52148=CARTESIAN_POINT ( 'NONE',  ( 6.449999999999928235, 2.500000000000000000, 2.511473670974873507 ) ) ;
#52149=FACE_OUTER_BOUND ( 'NONE', #119153, .T. ) ;
#52150=FACE_BOUND ( 'NONE', #53558, .T. ) ;
#52151=ORIENTED_EDGE ( 'NONE', *, *, #24614, .F. ) ;
#52153=CIRCLE ( 'NONE', #12425, 0.1000000000000002554 ) ;
#52154=FACE_OUTER_BOUND ( 'NONE', #125038, .T. ) ;
#52155=PLANE ( 'NONE',  #127474 ) ;
#52156=EDGE_CURVE ( 'NONE', #47060, #42654, #52524, .T. ) ;
#52157=DIRECTION ( 'NONE',  ( 0.000000000000000000, 0.000000000000000000, -1.000000000000000000 ) ) ;
#52158=DIRECTION ( 'NONE',  ( -4.274815082592931898E-19, -0.9999939076577903929, -0.003490651415223739937 ) ) ;
#52160=CIRCLE ( 'NONE', #85599, 0.06509327318403745899 ) ;
#52161=CARTESIAN_POINT ( 'NONE',  ( 11.84999999999990727, 2.500000000000000000, 6.248780366869520542 ) ) ;
#52162=CARTESIAN_POINT ( 'NONE',  ( 12.69999999999989804, 2.500000000000000000, 0.3464101615137735735 ) ) ;
#52163=CONICAL_SURFACE ( 'NONE', #12440, 0.1000000000000002554, 0.003490658503988666988 ) ;
#52164=CIRCLE ( 'NONE', #6175, 0.06509327318403745899 ) ;
#52165=EDGE_LOOP ( 'NONE', ( #74430, #36069 ) ) ;
#52166=ORIENTED_EDGE ( 'NONE', *, *, #33888, .T. ) ;
#52167=VERTEX_POINT ( 'NONE', #57216 ) ;
#52168=ORIENTED_EDGE ( 'NONE', *, *, #55600, .T. ) ;
#52169=EDGE_LOOP ( 'NONE', ( #97257, #80397 ) ) ;
#52170=LINE ( 'NONE', #80348, #87792 ) ;
#52171=AXIS2_PLACEMENT_3D ( 'NONE', #91145, #79403, #49957 ) ;
#52172=LINE ( 'NONE', #31890, #27810 ) ;
#52173=ORIENTED_EDGE ( 'NONE', *, *, #118537, .T. ) ;
#52174=FACE_BOUND ( 'NONE', #123127, .T. ) ;
#52175=DIRECTION ( 'NONE',  ( -0.000000000000000000, -1.000000000000000000, -0.000000000000000000 ) ) ;
#52177=EDGE_LOOP ( 'NONE', ( #17609, #2516 ) ) ;
#52178=FACE_OUTER_BOUND ( 'NONE', #41227, .T. ) ;
#52179=CARTESIAN_POINT ( 'NONE',  ( 5.849999999999933920, 2.500000000000000000, -2.265063509461101798 ) ) ;
#52180=CARTESIAN_POINT ( 'NONE',  ( 7.899999999999924860, 2.500000000000000000, 4.330127018922196314 ) ) ;
#52181=ORIENTED_EDGE ( 'NONE', *, *, #119539, .T. ) ;
#52182=CARTESIAN_POINT ( 'NONE',  ( 3.349999999999945466, 2.500000000000000000, -2.857883832488653741 ) ) ;
#52183=ORIENTED_EDGE ( 'NONE', *, *, #236, .F. ) ;
#52184=ORIENTED_EDGE ( 'NONE', *, *, #78366, .F. ) ;
#52185=ORIENTED_EDGE ( 'NONE', *, *, #54070, .T. ) ;
#52186=VECTOR ( 'NONE', #99033, 1000.000000000000000 ) ;
#52187=DIRECTION ( 'NONE',  ( -0.000000000000000000, 1.000000000000000000, -0.000000000000000000 ) ) ;
#52188=FACE_OUTER_BOUND ( 'NONE', #100938, .T. ) ;
#52189=ORIENTED_EDGE ( 'NONE', *, *, #62285, .F. ) ;
#52190=DIRECTION ( 'NONE',  ( 0.000000000000000000, 0.000000000000000000, 1.000000000000000000 ) ) ;
#52191=AXIS2_PLACEMENT_3D ( 'NONE', #23797, #44071, #83978 ) ;
#52192=EDGE_CURVE ( 'NONE', #126749, #93502, #110994, .T. ) ;
#52193=DIRECTION ( 'NONE',  ( 0.000000000000000000, 1.000000000000000000, 0.000000000000000000 ) ) ;
#52194=CARTESIAN_POINT ( 'NONE',  ( 0.1999999999999571565, 2.500000000000000000, 4.083716857408420609 ) ) ;
#52195=DIRECTION ( 'NONE',  ( 0.000000000000000000, 0.000000000000000000, 1.000000000000000000 ) ) ;
#52197=ORIENTED_EDGE ( 'NONE', *, *, #100282, .T. ) ;
#52198=EDGE_CURVE ( 'NONE', #84669, #112250, #54561, .T. ) ;
#52199=DIRECTION ( 'NONE',  ( 0.000000000000000000, -1.000000000000000000, 0.000000000000000000 ) ) ;
#52201=CONICAL_SURFACE ( 'NONE', #123222, 0.1000000000000002554, 0.003490658503988666988 ) ;
#52202=EDGE_LOOP ( 'NONE', ( #111258, #114077, #29061, #16288 ) ) ;
#52203=LINE ( 'NONE', #62029, #93071 ) ;
#52205=CIRCLE ( 'NONE', #29235, 0.06509327318403745899 ) ;
#52206=ORIENTED_EDGE ( 'NONE', *, *, #86096, .T. ) ;
#52207=DIRECTION ( 'NONE',  ( -0.000000000000000000, 1.000000000000000000, -0.000000000000000000 ) ) ;
#52208=EDGE_LOOP ( 'NONE', ( #2816, #67146 ) ) ;
#52209=FACE_OUTER_BOUND ( 'NONE', #3183, .T. ) ;
#52210=CARTESIAN_POINT ( 'NONE',  ( 10.39999999999991509, 2.500000000000000000, 0.6928203230275494784 ) ) ;
#52211=EDGE_CURVE ( 'NONE', #53342, #118322, #113158, .T. ) ;
#52212=ADVANCED_FACE ( 'NONE', ( #96477 ), #25317, .T. ) ;
#52213=CARTESIAN_POINT ( 'NONE',  ( 12.69999999999990337, 12.50000000000000000, 4.048810130592458201 ) ) ;
#52214=EDGE_CURVE ( 'NONE', #62130, #68394, #128572, .T. ) ;
#52215=CARTESIAN_POINT ( 'NONE',  ( -4.550000000000022915, 12.50000000000000000, 2.165063509461097713 ) ) ;
#52216=ADVANCED_FACE ( 'NONE', ( #38236 ), #50465, .T. ) ;
#52218=AXIS2_PLACEMENT_3D ( 'NONE', #43321, #114612, #64230 ) ;
#52219=ORIENTED_EDGE ( 'NONE', *, *, #100494, .F. ) ;
#52220=ORIENTED_EDGE ( 'NONE', *, *, #27070, .T. ) ;
#52221=AXIS2_PLACEMENT_3D ( 'NONE', #124563, #74812, #122627 ) ;
#52222=DIRECTION ( 'NONE',  ( -0.000000000000000000, 1.000000000000000000, -0.000000000000000000 ) ) ;
#52223=DIRECTION ( 'NONE',  ( 0.000000000000000000, 0.000000000000000000, -1.000000000000000000 ) ) ;
#52224=DIRECTION ( 'NONE',  ( 0.000000000000000000, 0.000000000000000000, -1.000000000000000000 ) ) ;
#52225=ORIENTED_EDGE ( 'NONE', *, *, #70323, .F. ) ;
#52226=VERTEX_POINT ( 'NONE', #29067 ) ;
#52227=ORIENTED_EDGE ( 'NONE', *, *, #124426, .T. ) ;
#52228=EDGE_CURVE ( 'NONE', #86441, #14402, #10669, .T. ) ;
#52229=FACE_OUTER_BOUND ( 'NONE', #25841, .T. ) ;
#52230=CIRCLE ( 'NONE', #8383, 0.06509327318403745899 ) ;
#52231=ORIENTED_EDGE ( 'NONE', *, *, #30771, .F. ) ;
#52232=LINE ( 'NONE', #91502, #94657 ) ;
#52233=DIRECTION ( 'NONE',  ( 0.000000000000000000, 1.000000000000000000, 0.000000000000000000 ) ) ;
#52234=DIRECTION ( 'NONE',  ( 0.000000000000000000, 1.000000000000000000, 0.000000000000000000 ) ) ;
#52235=ORIENTED_EDGE ( 'NONE', *, *, #60088, .T. ) ;
#52236=DIRECTION ( 'NONE',  ( 0.000000000000000000, 0.000000000000000000, 1.000000000000000000 ) ) ;
#52237=DIRECTION ( 'NONE',  ( 0.000000000000000000, 0.000000000000000000, 1.000000000000000000 ) ) ;
#52238=CARTESIAN_POINT ( 'NONE',  ( -8.350000000000013856, 2.500000000000000000, 2.065063509461097624 ) ) ;
#52239=CIRCLE ( 'NONE', #127448, 0.06509327318403743123 ) ;
#52240=DIRECTION ( 'NONE',  ( -0.000000000000000000, -1.000000000000000000, -0.000000000000000000 ) ) ;
#52241=LINE ( 'NONE', #50960, #26988 ) ;
#52242=ORIENTED_EDGE ( 'NONE', *, *, #57458, .F. ) ;
#52243=PLANE ( 'NONE',  #57133 ) ;
#52244=CARTESIAN_POINT ( 'NONE',  ( 23.99354682433153130, -2.839181451644544385, 2.508508607398769907 ) ) ;
#52245=VERTEX_POINT ( 'NONE', #91192 ) ;
#52246=ORIENTED_EDGE ( 'NONE', *, *, #52949, .T. ) ;
#52247=EDGE_CURVE ( 'NONE', #11408, #126604, #67158, .T. ) ;
#52249=CARTESIAN_POINT ( 'NONE',  ( 8.149999999999923972, 2.500000000000000000, -6.148780366869526226 ) ) ;
#52250=DIRECTION ( 'NONE',  ( -0.000000000000000000, 1.000000000000000000, -0.000000000000000000 ) ) ;
#52251=DIRECTION ( 'NONE',  ( 0.000000000000000000, 0.000000000000000000, 1.000000000000000000 ) ) ;
#52252=CARTESIAN_POINT ( 'NONE',  ( 5.399999999999932854, 2.500000000000000000, 3.737306695894644371 ) ) ;
#52253=DIRECTION ( 'NONE',  ( 0.000000000000000000, 0.000000000000000000, 1.000000000000000000 ) ) ;
#52254=PLANE ( 'NONE',  #105511 ) ;
#52255=CARTESIAN_POINT ( 'NONE',  ( 9.549999999999915445, 2.500000000000000000, 6.495190528383297135 ) ) ;
#52256=ADVANCED_FACE ( 'NONE', ( #21822 ), #41472, .T. ) ;
#52257=ADVANCED_FACE ( 'NONE', ( #30361 ), #48319, .T. ) ;
#52258=DIRECTION ( 'NONE',  ( 0.000000000000000000, 0.000000000000000000, 1.000000000000000000 ) ) ;
#52259=ORIENTED_EDGE ( 'NONE', *, *, #89963, .T. ) ;
#52260=ORIENTED_EDGE ( 'NONE', *, *, #96781, .F. ) ;
#52261=ADVANCED_FACE ( 'NONE', ( #61088 ), #19053, .T. ) ;
#52262=AXIS2_PLACEMENT_3D ( 'NONE', #69699, #51371, #129295 ) ;
#52263=ORIENTED_EDGE ( 'NONE', *, *, #79473, .F. ) ;
#52264=EDGE_LOOP ( 'NONE', ( #87127, #122172, #34016, #55217 ) ) ;
#52265=ADVANCED_FACE ( 'NONE', ( #121296 ), #65118, .T. ) ;
#52266=FACE_OUTER_BOUND ( 'NONE', #108873, .T. ) ;
#52267=DIRECTION ( 'NONE',  ( 0.000000000000000000, 0.000000000000000000, 1.000000000000000000 ) ) ;
#52268=ADVANCED_FACE ( 'NONE', ( #101006 ), #69323, .T. ) ;
#52269=CONICAL_SURFACE ( 'NONE', #29288, 0.09999999999999999167, 0.003490658503988666988 ) ;
#52270=VECTOR ( 'NONE', #65488, 1000.000000000000000 ) ;
#52271=EDGE_LOOP ( 'NONE', ( #62070, #65321, #33209, #78970 ) ) ;
#52272=ADVANCED_FACE ( 'NONE', ( #2157 ), #29626, .T. ) ;
#52273=CARTESIAN_POINT ( 'NONE',  ( -5.850000000000019185, 2.500000000000000000, 6.495190528383297135 ) ) ;
#52274=EDGE_CURVE ( 'NONE', #91490, #48067, #51924, .T. ) ;
#52275=DIRECTION ( 'NONE',  ( 0.000000000000000000, -0.000000000000000000, 1.000000000000000000 ) ) ;
#52276=DIRECTION ( 'NONE',  ( -0.000000000000000000, 1.000000000000000000, -0.000000000000000000 ) ) ;
#52277=ORIENTED_EDGE ( 'NONE', *, *, #38969, .F. ) ;
#52278=CARTESIAN_POINT ( 'NONE',  ( -8.300000000000011369, 2.500000000000000000, -4.330127018922201643 ) ) ;
#52279=EDGE_CURVE ( 'NONE', #83089, #81926, #32305, .T. ) ;
#52280=DIRECTION ( 'NONE',  ( 0.000000000000000000, 0.000000000000000000, 1.000000000000000000 ) ) ;
#52281=EDGE_LOOP ( 'NONE', ( #42552, #41889 ) ) ;
#52282=ORIENTED_EDGE ( 'NONE', *, *, #63931, .F. ) ;
#52283=ORIENTED_EDGE ( 'NONE', *, *, #68048, .F. ) ;
#52284=ORIENTED_EDGE ( 'NONE', *, *, #85625, .F. ) ;
#52285=DIRECTION ( 'NONE',  ( 0.000000000000000000, 0.000000000000000000, 1.000000000000000000 ) ) ;
#52286=CARTESIAN_POINT ( 'NONE',  ( 7.299999999999926104, 2.500000000000000000, -0.3464101615137782364 ) ) ;
#52287=CARTESIAN_POINT ( 'NONE',  ( 5.799999999999933209, 2.500000000000000000, -2.385244779468109755E-15 ) ) ;
#52288=DIRECTION ( 'NONE',  ( 0.000000000000000000, 0.000000000000000000, 1.000000000000000000 ) ) ;
#52289=AXIS2_PLACEMENT_3D ( 'NONE', #25482, #92963, #24215 ) ;
#52290=ORIENTED_EDGE ( 'NONE', *, *, #96371, .T. ) ;
#52291=AXIS2_PLACEMENT_3D ( 'NONE', #14018, #113521, #45444 ) ;
#52293=ORIENTED_EDGE ( 'NONE', *, *, #54873, .T. ) ;
#52294=CARTESIAN_POINT ( 'NONE',  ( -6.250000000000021316, 2.500000000000000000, -5.702370205355749455 ) ) ;
#52295=CARTESIAN_POINT ( 'NONE',  ( 15.79999999999989058, 2.500000000000000000, -0.1000000000000023925 ) ) ;
#52296=DIRECTION ( 'NONE',  ( 0.000000000000000000, 1.000000000000000000, 0.000000000000000000 ) ) ;
#52297=DIRECTION ( 'NONE',  ( 0.000000000000000000, 0.000000000000000000, 1.000000000000000000 ) ) ;
#52298=VERTEX_POINT ( 'NONE', #72210 ) ;
#52299=ORIENTED_EDGE ( 'NONE', *, *, #82251, .T. ) ;
#52300=VERTEX_POINT ( 'NONE', #112131 ) ;
#52301=DIRECTION ( 'NONE',  ( -4.274815082592931898E-19, -0.9999939076577903929, -0.003490651415223739937 ) ) ;
#52302=DIRECTION ( 'NONE',  ( 0.000000000000000000, 1.000000000000000000, 0.000000000000000000 ) ) ;
#52303=CARTESIAN_POINT ( 'NONE',  ( 9.149999999999915090, 2.500000000000000000, 6.595190528383296780 ) ) ;
#52304=FACE_BOUND ( 'NONE', #90334, .T. ) ;
#52305=CARTESIAN_POINT ( 'NONE',  ( 1.699999999999951994, 12.50000000000000000, -4.330127018922201643 ) ) ;
#52306=CARTESIAN_POINT ( 'NONE',  ( -4.800000000000024691, 12.50000000000000000, 4.676537180435972552 ) ) ;
#52307=LINE ( 'NONE', #61498, #89635 ) ;
#52308=AXIS2_PLACEMENT_3D ( 'NONE', #28944, #79339, #100258 ) ;
#52309=CIRCLE ( 'NONE', #89859, 0.06509327318403741736 ) ;
#52310=EDGE_CURVE ( 'NONE', #61474, #113589, #4555, .T. ) ;
#52311=DIRECTION ( 'NONE',  ( 0.000000000000000000, 0.000000000000000000, 1.000000000000000000 ) ) ;
#52312=DIRECTION ( 'NONE',  ( -0.000000000000000000, -1.000000000000000000, -0.000000000000000000 ) ) ;
#52313=LINE ( 'NONE', #32700, #19765 ) ;
#52314=ORIENTED_EDGE ( 'NONE', *, *, #89115, .T. ) ;
#52315=CONICAL_SURFACE ( 'NONE', #64915, 0.09999999999999999167, 0.003490658503988666988 ) ;
#52316=CARTESIAN_POINT ( 'NONE',  ( 8.149999999999923972, 2.500000000000000000, -6.048780366869526581 ) ) ;
#52317=DIRECTION ( 'NONE',  ( 0.000000000000000000, 0.000000000000000000, 1.000000000000000000 ) ) ;
#52318=AXIS2_PLACEMENT_3D ( 'NONE', #5922, #85785, #36060 ) ;
#52319=ORIENTED_EDGE ( 'NONE', *, *, #12389, .T. ) ;
#52321=CARTESIAN_POINT ( 'NONE',  ( 4.149999999999941735, 12.50000000000000000, -1.407149913249512663 ) ) ;
#52322=EDGE_CURVE ( 'NONE', #98563, #22598, #120653, .T. ) ;
#52323=CARTESIAN_POINT ( 'NONE',  ( 9.349999999999919709, 2.500000000000000000, -6.841600689897078702 ) ) ;
#52324=FACE_BOUND ( 'NONE', #62984, .T. ) ;
#52325=DIRECTION ( 'NONE',  ( 0.000000000000000000, 0.000000000000000000, 1.000000000000000000 ) ) ;
#52326=EDGE_LOOP ( 'NONE', ( #16171, #80839 ) ) ;
#52327=DIRECTION ( 'NONE',  ( 0.000000000000000000, 0.000000000000000000, 1.000000000000000000 ) ) ;
#52328=CARTESIAN_POINT ( 'NONE',  ( 0.1999999999999627909, 2.500000000000000000, 0.3464101615137758494 ) ) ;
#52329=ORIENTED_EDGE ( 'NONE', *, *, #4311, .F. ) ;
#52330=FACE_OUTER_BOUND ( 'NONE', #57973, .T. ) ;
#52331=DIRECTION ( 'NONE',  ( 0.000000000000000000, -0.000000000000000000, 1.000000000000000000 ) ) ;
#52332=AXIS2_PLACEMENT_3D ( 'NONE', #39702, #27258, #48198 ) ;
#52333=ORIENTED_EDGE ( 'NONE', *, *, #129595, .T. ) ;
#52334=CARTESIAN_POINT ( 'NONE',  ( 1.649999999999951950, 12.50000000000000000, -7.188010851410854052 ) ) ;
#52336=CARTESIAN_POINT ( 'NONE',  ( 9.999999999999914735, 2.500000000000000000, 0.6928203230275494784 ) ) ;
#52337=EDGE_LOOP ( 'NONE', ( #125291, #24258 ) ) ;
#52338=ADVANCED_FACE ( 'NONE', ( #11343 ), #42099, .T. ) ;
#52339=CARTESIAN_POINT ( 'NONE',  ( 1.849999999999950573, 2.500000000000000000, -1.818653347947326138 ) ) ;
#52340=CONICAL_SURFACE ( 'NONE', #119241, 0.09999999999999982514, 0.003490658503988666988 ) ;
#52341=VECTOR ( 'NONE', #59258, 1000.000000000000000 ) ;
#52342=CARTESIAN_POINT ( 'NONE',  ( 11.04999999999991012, 2.500000000000000000, -1.718653347947326049 ) ) ;
#52343=DIRECTION ( 'NONE',  ( 0.000000000000000000, 1.000000000000000000, 0.000000000000000000 ) ) ;
#52344=ORIENTED_EDGE ( 'NONE', *, *, #95085, .F. ) ;
#52345=ORIENTED_EDGE ( 'NONE', *, *, #108524, .F. ) ;
#52346=CARTESIAN_POINT ( 'NONE',  ( -2.499999999999996003, 2.500000000000000000, -2.276824562219559311E-15 ) ) ;
#52347=EDGE_CURVE ( 'NONE', #118274, #80116, #6606, .T. ) ;
#52348=EDGE_LOOP ( 'NONE', ( #108075, #2776 ) ) ;
#52349=CARTESIAN_POINT ( 'NONE',  ( 9.149999999999916866, 2.500000000000000000, -2.857883832488653741 ) ) ;
#52350=DIRECTION ( 'NONE',  ( 0.000000000000000000, 0.000000000000000000, 1.000000000000000000 ) ) ;
#52351=CARTESIAN_POINT ( 'NONE',  ( -2.100000000000034728, 12.50000000000000000, 4.330127018922196314 ) ) ;
#52352=EDGE_LOOP ( 'NONE', ( #6048, #128255, #106246, #114048 ) ) ;
#52353=LINE ( 'NONE', #81805, #26559 ) ;
#52354=DIRECTION ( 'NONE',  ( 0.000000000000000000, 1.000000000000000000, 0.000000000000000000 ) ) ;
#52355=CARTESIAN_POINT ( 'NONE',  ( 13.09999999999990195, 2.500000000000000000, 4.676537180435972552 ) ) ;
#52356=EDGE_CURVE ( 'NONE', #19644, #16889, #48412, .T. ) ;
#52357=EDGE_CURVE ( 'NONE', #46368, #110642, #119507, .T. ) ;
#52358=DIRECTION ( 'NONE',  ( -0.000000000000000000, -1.000000000000000000, -0.000000000000000000 ) ) ;
#52359=DIRECTION ( 'NONE',  ( -0.000000000000000000, -1.000000000000000000, -0.000000000000000000 ) ) ;
#52360=EDGE_CURVE ( 'NONE', #92622, #36126, #23350, .T. ) ;
#52361=ADVANCED_FACE ( 'NONE', ( #43399 ), #125783, .T. ) ;
#52362=ADVANCED_FACE ( 'NONE', ( #4089 ), #42154, .T. ) ;
#52363=PLANE ( 'NONE',  #45314 ) ;
#52364=EDGE_LOOP ( 'NONE', ( #21764, #127613, #36215, #14151 ) ) ;
#52365=VERTEX_POINT ( 'NONE', #84595 ) ;
#52366=DIRECTION ( 'NONE',  ( 0.000000000000000000, -0.000000000000000000, 1.000000000000000000 ) ) ;
#52367=ORIENTED_EDGE ( 'NONE', *, *, #127433, .T. ) ;
#52368=DIRECTION ( 'NONE',  ( 0.000000000000000000, 1.000000000000000000, 0.000000000000000000 ) ) ;
#52369=ORIENTED_EDGE ( 'NONE', *, *, #67577, .F. ) ;
#52370=EDGE_LOOP ( 'NONE', ( #100921, #86266, #111536, #2364 ) ) ;
#52371=ORIENTED_EDGE ( 'NONE', *, *, #71860, .F. ) ;
#52372=EDGE_CURVE ( 'NONE', #32930, #122361, #13258, .T. ) ;
#52373=CARTESIAN_POINT ( 'NONE',  ( 0.3999999999999559464, 12.50000000000000000, -4.395220292106239768 ) ) ;
#52374=ADVANCED_FACE ( 'NONE', ( #83932 ), #4714, .T. ) ;
#52375=AXIS2_PLACEMENT_3D ( 'NONE', #18442, #28268, #86534 ) ;
#52376=DIRECTION ( 'NONE',  ( 0.000000000000000000, 0.000000000000000000, -1.000000000000000000 ) ) ;
#52377=EDGE_CURVE ( 'NONE', #103313, #114323, #113249, .T. ) ;
#52378=AXIS2_PLACEMENT_3D ( 'NONE', #93442, #83632, #123531 ) ;
#52379=DIRECTION ( 'NONE',  ( 0.000000000000000000, 0.000000000000000000, 1.000000000000000000 ) ) ;
#52380=DIRECTION ( 'NONE',  ( 0.000000000000000000, -0.000000000000000000, 1.000000000000000000 ) ) ;
#52381=DIRECTION ( 'NONE',  ( 0.000000000000000000, 1.000000000000000000, 0.000000000000000000 ) ) ;
#52382=DIRECTION ( 'NONE',  ( -0.000000000000000000, -1.000000000000000000, -0.000000000000000000 ) ) ;
#52383=DIRECTION ( 'NONE',  ( -4.274815082592931898E-19, -0.9999939076577903929, -0.003490651415223739937 ) ) ;
#52384=FACE_OUTER_BOUND ( 'NONE', #90890, .T. ) ;
#52385=DIRECTION ( 'NONE',  ( -0.000000000000000000, -1.000000000000000000, -0.000000000000000000 ) ) ;
#52386=CONICAL_SURFACE ( 'NONE', #125535, 0.1000000000000002554, 0.003490658503988666988 ) ;
#52387=ORIENTED_EDGE ( 'NONE', *, *, #48389, .T. ) ;
#52388=DIRECTION ( 'NONE',  ( 0.000000000000000000, 0.000000000000000000, 1.000000000000000000 ) ) ;
#52389=ORIENTED_EDGE ( 'NONE', *, *, #114389, .T. ) ;
#52390=EDGE_LOOP ( 'NONE', ( #15828, #58530 ) ) ;
#52391=DIRECTION ( 'NONE',  ( 0.000000000000000000, 0.000000000000000000, 1.000000000000000000 ) ) ;
#52392=DIRECTION ( 'NONE',  ( 0.000000000000000000, 0.000000000000000000, -1.000000000000000000 ) ) ;
#52393=CARTESIAN_POINT ( 'NONE',  ( 1.649999999999949729, 2.500000000000000000, 5.802370205355744659 ) ) ;
#52394=AXIS2_PLACEMENT_3D ( 'NONE', #41980, #93654, #81258 ) ;
#52395=CARTESIAN_POINT ( 'NONE',  ( 10.59999999999991260, 12.50000000000000000, -0.2813168883297409439 ) ) ;
#52396=AXIS2_PLACEMENT_3D ( 'NONE', #35251, #83696, #26708 ) ;
#52398=DIRECTION ( 'NONE',  ( 0.000000000000000000, 0.000000000000000000, 1.000000000000000000 ) ) ;
#52399=CARTESIAN_POINT ( 'NONE',  ( -4.800000000000022915, 12.50000000000000000, -0.3464101615137783474 ) ) ;
#52400=DIRECTION ( 'NONE',  ( 0.000000000000000000, 0.000000000000000000, -1.000000000000000000 ) ) ;
#52401=ORIENTED_EDGE ( 'NONE', *, *, #44369, .F. ) ;
#52402=AXIS2_PLACEMENT_3D ( 'NONE', #98651, #129451, #39774 ) ;
#52403=ORIENTED_EDGE ( 'NONE', *, *, #3486, .F. ) ;
#52404=ORIENTED_EDGE ( 'NONE', *, *, #51792, .F. ) ;
#52405=AXIS2_PLACEMENT_3D ( 'NONE', #11747, #90959, #62160 ) ;
#52406=ORIENTED_EDGE ( 'NONE', *, *, #33951, .F. ) ;
#52407=ADVANCED_FACE ( 'NONE', ( #54479 ), #94399, .T. ) ;
#52408=EDGE_LOOP ( 'NONE', ( #1569, #20747, #64247, #123419 ) ) ;
#52409=CARTESIAN_POINT ( 'NONE',  ( 15.19999999999989093, 12.50000000000000000, 0.3464101615137735735 ) ) ;
#52410=CARTESIAN_POINT ( 'NONE',  ( -8.350000000000012079, 12.50000000000000000, 1.537336459617582918 ) ) ;
#52411=EDGE_CURVE ( 'NONE', #60152, #2388, #21214, .T. ) ;
#52412=DIRECTION ( 'NONE',  ( 0.000000000000000000, 1.000000000000000000, 0.000000000000000000 ) ) ;
#52413=DIRECTION ( 'NONE',  ( 0.000000000000000000, 0.000000000000000000, -1.000000000000000000 ) ) ;
#52414=EDGE_CURVE ( 'NONE', #49812, #60985, #73528, .T. ) ;
#52415=DIRECTION ( 'NONE',  ( 0.000000000000000000, -0.000000000000000000, 1.000000000000000000 ) ) ;
#52416=ORIENTED_EDGE ( 'NONE', *, *, #124157, .T. ) ;
#52417=DIRECTION ( 'NONE',  ( 0.000000000000000000, 0.000000000000000000, 1.000000000000000000 ) ) ;
#52418=FACE_OUTER_BOUND ( 'NONE', #56507, .T. ) ;
#52419=DIRECTION ( 'NONE',  ( 0.000000000000000000, 0.000000000000000000, -1.000000000000000000 ) ) ;
#52420=EDGE_CURVE ( 'NONE', #5314, #69112, #56791, .T. ) ;
#52422=ORIENTED_EDGE ( 'NONE', *, *, #87419, .F. ) ;
#52423=ORIENTED_EDGE ( 'NONE', *, *, #93776, .T. ) ;
#52424=ORIENTED_EDGE ( 'NONE', *, *, #68329, .T. ) ;
#52425=AXIS2_PLACEMENT_3D ( 'NONE', #3930, #21650, #52391 ) ;
#52426=DIRECTION ( 'NONE',  ( 0.000000000000000000, -0.9999939076577903929, 0.003490651415223739937 ) ) ;
#52427=AXIS2_PLACEMENT_3D ( 'NONE', #121307, #61760, #51933 ) ;
#52428=AXIS2_PLACEMENT_3D ( 'NONE', #81528, #26477, #124020 ) ;
#52429=EDGE_LOOP ( 'NONE', ( #126686, #84987 ) ) ;
#52430=DIRECTION ( 'NONE',  ( 0.000000000000000000, 1.000000000000000000, 0.000000000000000000 ) ) ;
#52431=CARTESIAN_POINT ( 'NONE',  ( -1.250000000000036193, 2.500000000000000000, 1.372243186433545370 ) ) ;
#52432=AXIS2_PLACEMENT_3D ( 'NONE', #88492, #76752, #17815 ) ;
#52433=CIRCLE ( 'NONE', #27376, 0.09999999999999982514 ) ;
#52434=ORIENTED_EDGE ( 'NONE', *, *, #47318, .F. ) ;
#52435=DIRECTION ( 'NONE',  ( 0.000000000000000000, 0.000000000000000000, 1.000000000000000000 ) ) ;
#52436=CARTESIAN_POINT ( 'NONE',  ( 0.7999999999999612976, 2.500000000000000000, -1.084202172485504434E-16 ) ) ;
#52437=DIRECTION ( 'NONE',  ( -0.000000000000000000, -1.000000000000000000, -0.000000000000000000 ) ) ;
#52438=EDGE_CURVE ( 'NONE', #24620, #11460, #64934, .T. ) ;
#52439=FACE_OUTER_BOUND ( 'NONE', #105227, .T. ) ;
#52440=DIRECTION ( 'NONE',  ( 0.000000000000000000, 0.000000000000000000, 1.000000000000000000 ) ) ;
#52441=ORIENTED_EDGE ( 'NONE', *, *, #27350, .T. ) ;
#52442=VERTEX_POINT ( 'NONE', #36142 ) ;
#52443=CARTESIAN_POINT ( 'NONE',  ( -1.050000000000038236, 12.50000000000000000, -1.753560074763288679 ) ) ;
#52444=CARTESIAN_POINT ( 'NONE',  ( -7.900000000000011013, 2.500000000000000000, 5.022947341949748790 ) ) ;
#52445=DIRECTION ( 'NONE',  ( 0.000000000000000000, 0.000000000000000000, 1.000000000000000000 ) ) ;
#52446=DIRECTION ( 'NONE',  ( 0.000000000000000000, -0.9999939076577903929, 0.003490651415223739937 ) ) ;
#52447=VERTEX_POINT ( 'NONE', #105527 ) ;
#52448=CIRCLE ( 'NONE', #92163, 0.1000000000000002554 ) ;
#52449=EDGE_CURVE ( 'NONE', #118122, #76584, #112776, .T. ) ;
#52450=ORIENTED_EDGE ( 'NONE', *, *, #76730, .T. ) ;
#52451=LINE ( 'NONE', #70174, #33365 ) ;
#52452=DIRECTION ( 'NONE',  ( 0.000000000000000000, 0.000000000000000000, 1.000000000000000000 ) ) ;
#52453=CARTESIAN_POINT ( 'NONE',  ( 13.54999999999989946, 2.500000000000000000, 2.611473670974873151 ) ) ;
#52454=CARTESIAN_POINT ( 'NONE',  ( -8.150000000000012790, 12.50000000000000000, -2.576566944158915184 ) ) ;
#52455=VERTEX_POINT ( 'NONE', #114060 ) ;
#52456=CIRCLE ( 'NONE', #125608, 0.06509327318403745899 ) ;
#52457=CARTESIAN_POINT ( 'NONE',  ( -12.89999999999999147, 2.500000000000000000, 3.637306695894644726 ) ) ;
#52458=CIRCLE ( 'NONE', #90100, 0.06509327318403745899 ) ;
#52459=CARTESIAN_POINT ( 'NONE',  ( -5.400000000000023448, 2.500000000000000000, -4.922947341949753586 ) ) ;
#52460=ORIENTED_EDGE ( 'NONE', *, *, #65468, .T. ) ;
#52461=DIRECTION ( 'NONE',  ( 0.000000000000000000, 0.000000000000000000, -1.000000000000000000 ) ) ;
#52462=EDGE_CURVE ( 'NONE', #101658, #16388, #17071, .T. ) ;
#52463=ORIENTED_EDGE ( 'NONE', *, *, #40588, .T. ) ;
#52464=CIRCLE ( 'NONE', #37897, 0.09999999999999982514 ) ;
#52465=FACE_OUTER_BOUND ( 'NONE', #70715, .T. ) ;
#52466=AXIS2_PLACEMENT_3D ( 'NONE', #67499, #97631, #106169 ) ;
#52467=ORIENTED_EDGE ( 'NONE', *, *, #98170, .T. ) ;
#52468=CARTESIAN_POINT ( 'NONE',  ( 6.649999999999929301, 12.50000000000000000, -2.165063509461101710 ) ) ;
#52469=DIRECTION ( 'NONE',  ( -0.000000000000000000, -1.000000000000000000, -0.000000000000000000 ) ) ;
#52470=EDGE_LOOP ( 'NONE', ( #117757, #59300 ) ) ;
#52471=ADVANCED_FACE ( 'NONE', ( #104858 ), #14923, .T. ) ;
#52472=ORIENTED_EDGE ( 'NONE', *, *, #18127, .F. ) ;
#52473=DIRECTION ( 'NONE',  ( -0.000000000000000000, -1.000000000000000000, -0.000000000000000000 ) ) ;
#52474=CIRCLE ( 'NONE', #121516, 0.06509327318403745899 ) ;
#52475=CARTESIAN_POINT ( 'NONE',  ( 9.599999999999914380, 12.50000000000000000, -3.572213422710612374 ) ) ;
#52477=CIRCLE ( 'NONE', #71262, 0.06509327318403745899 ) ;
#52478=LINE ( 'NONE', #41400, #103893 ) ;
#52479=CARTESIAN_POINT ( 'NONE',  ( 4.149999999999938183, 12.50000000000000000, 5.737276932171707422 ) ) ;
#52480=CARTESIAN_POINT ( 'NONE',  ( 12.89999999999990088, 2.500000000000000000, 4.330127018922196314 ) ) ;
#52481=DIRECTION ( 'NONE',  ( 0.000000000000000000, 0.000000000000000000, 1.000000000000000000 ) ) ;
#52482=DIRECTION ( 'NONE',  ( 0.000000000000000000, -0.000000000000000000, 1.000000000000000000 ) ) ;
#52483=CIRCLE ( 'NONE', #6484, 0.06509327318403745899 ) ;
#52484=ORIENTED_EDGE ( 'NONE', *, *, #24596, .T. ) ;
#52485=ADVANCED_FACE ( 'NONE', ( #73471 ), #81849, .T. ) ;
#52486=ORIENTED_EDGE ( 'NONE', *, *, #120257, .F. ) ;
#52487=CARTESIAN_POINT ( 'NONE',  ( -8.749999999999971578, 12.50000000000000000, 6.495190528383297135 ) ) ;
#52488=VERTEX_POINT ( 'NONE', #5379 ) ;
#52489=CIRCLE ( 'NONE', #106775, 0.1000000000000000056 ) ;
#52490=VECTOR ( 'NONE', #115644, 1000.000000000000000 ) ;
#52491=DIRECTION ( 'NONE',  ( -0.000000000000000000, -1.000000000000000000, -0.000000000000000000 ) ) ;
#52492=DIRECTION ( 'NONE',  ( 0.000000000000000000, 1.000000000000000000, 0.000000000000000000 ) ) ;
#52493=CARTESIAN_POINT ( 'NONE',  ( -2.700000000000030376, 12.50000000000000000, 4.048810130592458201 ) ) ;
#52494=EDGE_LOOP ( 'NONE', ( #92466, #39892, #72663, #38402 ) ) ;
#52496=FACE_BOUND ( 'NONE', #119718, .T. ) ;
#52497=EDGE_LOOP ( 'NONE', ( #73849, #76599 ) ) ;
#52498=DIRECTION ( 'NONE',  ( 0.000000000000000000, -0.9999939076577903929, 0.003490651415223739937 ) ) ;
#52499=CARTESIAN_POINT ( 'NONE',  ( 20.59313469514014017, -2.666874593322329456, 2.243770147468747034 ) ) ;
#52500=DIRECTION ( 'NONE',  ( -0.000000000000000000, -1.000000000000000000, -0.000000000000000000 ) ) ;
#52501=ADVANCED_FACE ( 'NONE', ( #63677 ), #13905, .T. ) ;
#52502=DIRECTION ( 'NONE',  ( -4.274815082592931898E-19, -0.9999939076577903929, -0.003490651415223739937 ) ) ;
#52504=CARTESIAN_POINT ( 'NONE',  ( -0.6000000000000383915, 2.500000000000000000, -4.676537180435977881 ) ) ;
#52505=CARTESIAN_POINT ( 'NONE',  ( 0.8499999999999553468, 2.500000000000000000, 2.065063509461097624 ) ) ;
#52506=DIRECTION ( 'NONE',  ( 0.000000000000000000, -0.9999939076577903929, 0.003490651415223739937 ) ) ;
#52507=EDGE_CURVE ( 'NONE', #104306, #75844, #94373, .T. ) ;
#52508=EDGE_CURVE ( 'NONE', #106389, #128383, #37950, .T. ) ;
#52509=CARTESIAN_POINT ( 'NONE',  ( 10.64999999999990976, 12.50000000000000000, -6.841600689897077814 ) ) ;
#52510=CARTESIAN_POINT ( 'NONE',  ( -3.350000000000028955, 2.500000000000000000, 7.188010851410848723 ) ) ;
#52511=EDGE_CURVE ( 'NONE', #94677, #21207, #7301, .T. ) ;
#52512=EDGE_CURVE ( 'NONE', #71164, #21407, #71378, .T. ) ;
#52513=CARTESIAN_POINT ( 'NONE',  ( -8.350000000000013856, 12.50000000000000000, 2.099970236277060032 ) ) ;
#52514=VERTEX_POINT ( 'NONE', #87797 ) ;
#52515=VERTEX_POINT ( 'NONE', #115982 ) ;
#52516=VERTEX_POINT ( 'NONE', #76706 ) ;
#52517=CARTESIAN_POINT ( 'NONE',  ( 11.84999999999990727, 2.500000000000000000, 6.148780366869520009 ) ) ;
#52518=ORIENTED_EDGE ( 'NONE', *, *, #122813, .T. ) ;
#52519=PLANE ( 'NONE',  #24661 ) ;
#52520=EDGE_CURVE ( 'NONE', #18680, #62169, #25405, .T. ) ;
#52521=CIRCLE ( 'NONE', #79706, 0.1000000000000002554 ) ;
#52522=CARTESIAN_POINT ( 'NONE',  ( -8.950000000000004619, 2.500000000000000000, 6.248780366869521430 ) ) ;
#52523=CIRCLE ( 'NONE', #75493, 0.1000000000000002554 ) ;
#52524=CIRCLE ( 'NONE', #62990, 0.1000000000000000472 ) ;
#52525=EDGE_CURVE ( 'NONE', #105322, #21282, #58883, .T. ) ;
#52526=ORIENTED_EDGE ( 'NONE', *, *, #64487, .F. ) ;
#52527=ORIENTED_EDGE ( 'NONE', *, *, #83125, .F. ) ;
#52528=EDGE_LOOP ( 'NONE', ( #20556, #96868, #72572, #80997 ) ) ;
#52529=ADVANCED_FACE ( 'NONE', ( #107452 ), #96326, .T. ) ;
#52530=DIRECTION ( 'NONE',  ( 0.000000000000000000, 1.000000000000000000, 0.000000000000000000 ) ) ;
#52531=ADVANCED_FACE ( 'NONE', ( #9257 ), #49203, .T. ) ;
#52532=AXIS2_PLACEMENT_3D ( 'NONE', #56295, #105413, #66758 ) ;
#52533=EDGE_CURVE ( 'NONE', #67175, #40177, #109030, .T. ) ;
#52534=CARTESIAN_POINT ( 'NONE',  ( 6.649999999999928413, 2.500000000000000000, 1.372243186433545370 ) ) ;
#52535=AXIS2_PLACEMENT_3D ( 'NONE', #99224, #46900, #78304 ) ;
#52536=CARTESIAN_POINT ( 'NONE',  ( 9.399999999999915090, 2.500000000000000000, -3.883716857408426648 ) ) ;
#52537=CARTESIAN_POINT ( 'NONE',  ( 87.50000000000001421, -3.975350567648449740, -6.360562287258772152 ) ) ;
#52538=FACE_OUTER_BOUND ( 'NONE', #86302, .T. ) ;
#52539=AXIS2_PLACEMENT_3D ( 'NONE', #105004, #114826, #84080 ) ;
#52540=DIRECTION ( 'NONE',  ( -0.000000000000000000, -1.000000000000000000, -0.000000000000000000 ) ) ;
#52541=EDGE_LOOP ( 'NONE', ( #814, #25669, #55556, #105154 ) ) ;
#52542=EDGE_CURVE ( 'NONE', #73050, #35098, #44387, .T. ) ;
#52543=DIRECTION ( 'NONE',  ( -0.000000000000000000, 1.000000000000000000, -0.000000000000000000 ) ) ;
#52544=ORIENTED_EDGE ( 'NONE', *, *, #68714, .F. ) ;
#52545=ORIENTED_EDGE ( 'NONE', *, *, #46770, .T. ) ;
#52546=ORIENTED_EDGE ( 'NONE', *, *, #94052, .T. ) ;
#52547=DIRECTION ( 'NONE',  ( -4.274815082592931898E-19, -0.9999939076577903929, -0.003490651415223739937 ) ) ;
#52548=ORIENTED_EDGE ( 'NONE', *, *, #76888, .F. ) ;
#52549=ORIENTED_EDGE ( 'NONE', *, *, #23226, .T. ) ;
#52550=ORIENTED_EDGE ( 'NONE', *, *, #121826, .T. ) ;
#52552=CARTESIAN_POINT ( 'NONE',  ( -12.69999999999999218, 2.500000000000000000, -4.776537180435974861 ) ) ;
#52553=CARTESIAN_POINT ( 'NONE',  ( 0.3999999999999619971, 12.50000000000000000, -1.084202172485504434E-16 ) ) ;
#52554=DIRECTION ( 'NONE',  ( 0.000000000000000000, -0.000000000000000000, 1.000000000000000000 ) ) ;
#52555=DIRECTION ( 'NONE',  ( -4.274815082592931898E-19, -0.9999939076577903929, -0.003490651415223739937 ) ) ;
#52556=CARTESIAN_POINT ( 'NONE',  ( -7.100000000000018296, 2.500000000000000000, -4.430127018922202176 ) ) ;
#52557=CIRCLE ( 'NONE', #25352, 0.06509327318403745899 ) ;
#52558=EDGE_LOOP ( 'NONE', ( #68671, #111488 ) ) ;
#52559=CARTESIAN_POINT ( 'NONE',  ( -11.24999999999996270, 12.50000000000000000, 2.099970236277060032 ) ) ;
#52561=CARTESIAN_POINT ( 'NONE',  ( 8.099999999999923261, 12.50000000000000000, -4.048810130592463530 ) ) ;
#52562=ORIENTED_EDGE ( 'NONE', *, *, #99969, .F. ) ;
#52563=LINE ( 'NONE', #40840, #61472 ) ;
#52564=ORIENTED_EDGE ( 'NONE', *, *, #17653, .F. ) ;
#52565=CIRCLE ( 'NONE', #121603, 0.06509327318403745899 ) ;
#52567=AXIS2_PLACEMENT_3D ( 'NONE', #28095, #7800, #109215 ) ;
#52568=EDGE_CURVE ( 'NONE', #33832, #125681, #25503, .T. ) ;
#52569=CARTESIAN_POINT ( 'NONE',  ( 0.7999999999999553024, 12.50000000000000000, -4.265033745738164406 ) ) ;
#52570=ADVANCED_FACE ( 'NONE', ( #98268 ), #102861, .T. ) ;
#52571=ORIENTED_EDGE ( 'NONE', *, *, #57561, .T. ) ;
#52572=ORIENTED_EDGE ( 'NONE', *, *, #123992, .F. ) ;
#52573=DIRECTION ( 'NONE',  ( -0.000000000000000000, -1.000000000000000000, -0.000000000000000000 ) ) ;
#52574=DIRECTION ( 'NONE',  ( 0.000000000000000000, -0.000000000000000000, 1.000000000000000000 ) ) ;
#52575=FACE_OUTER_BOUND ( 'NONE', #53595, .T. ) ;
#52576=CARTESIAN_POINT ( 'NONE',  ( -10.20000000000000462, 2.500000000000000000, 4.676537180435972552 ) ) ;
#52577=CIRCLE ( 'NONE', #73403, 0.06509327318403741736 ) ;
#52578=EDGE_CURVE ( 'NONE', #71646, #92201, #96598, .T. ) ;
#52579=CIRCLE ( 'NONE', #46224, 0.06509327318403745899 ) ;
#52580=DIRECTION ( 'NONE',  ( 0.000000000000000000, 0.000000000000000000, 1.000000000000000000 ) ) ;
#52581=ORIENTED_EDGE ( 'NONE', *, *, #63871, .T. ) ;
#52582=DIRECTION ( 'NONE',  ( -0.000000000000000000, -1.000000000000000000, -0.000000000000000000 ) ) ;
#52583=AXIS2_PLACEMENT_3D ( 'NONE', #71759, #92681, #42973 ) ;
#52584=AXIS2_PLACEMENT_3D ( 'NONE', #67083, #118794, #27829 ) ;
#52585=ORIENTED_EDGE ( 'NONE', *, *, #2567, .F. ) ;
#52586=CARTESIAN_POINT ( 'NONE',  ( -4.550000000000022915, 12.50000000000000000, 6.495190528383297135 ) ) ;
#52587=DIRECTION ( 'NONE',  ( -0.000000000000000000, 1.000000000000000000, -0.000000000000000000 ) ) ;
#52588=AXIS2_PLACEMENT_3D ( 'NONE', #29628, #28352, #69544 ) ;
#52589=AXIS2_PLACEMENT_3D ( 'NONE', #43562, #93289, #34391 ) ;
#52591=CARTESIAN_POINT ( 'NONE',  ( -3.950000000000024603, 2.500000000000000000, -2.411473670974877859 ) ) ;
#52592=DIRECTION ( 'NONE',  ( 0.000000000000000000, 0.000000000000000000, 1.000000000000000000 ) ) ;
#52593=CARTESIAN_POINT ( 'NONE',  ( -5.200000000000022382, 12.50000000000000000, 0.3464101615137735735 ) ) ;
#52594=CARTESIAN_POINT ( 'NONE',  ( 6.249999999999932498, 12.50000000000000000, 5.802370205355744659 ) ) ;
#52595=EDGE_LOOP ( 'NONE', ( #70906, #12002 ) ) ;
#52596=DIRECTION ( 'NONE',  ( 0.000000000000000000, 0.000000000000000000, 1.000000000000000000 ) ) ;
#52597=CARTESIAN_POINT ( 'NONE',  ( -10.84999999999999964, 2.500000000000000000, 2.757883832488649656 ) ) ;
#52598=FACE_OUTER_BOUND ( 'NONE', #55388, .T. ) ;
#52599=ORIENTED_EDGE ( 'NONE', *, *, #46519, .F. ) ;
#52600=ORIENTED_EDGE ( 'NONE', *, *, #117211, .F. ) ;
#52601=CARTESIAN_POINT ( 'NONE',  ( 5.649999999999932854, 2.500000000000000000, 1.818653347947321475 ) ) ;
#52603=EDGE_LOOP ( 'NONE', ( #41770, #103411 ) ) ;
#52604=VERTEX_POINT ( 'NONE', #89106 ) ;
#52605=DIRECTION ( 'NONE',  ( 0.000000000000000000, 0.000000000000000000, -1.000000000000000000 ) ) ;
#52607=VECTOR ( 'NONE', #91841, 1000.000000000000000 ) ;
#52608=EDGE_LOOP ( 'NONE', ( #91711, #116262, #78454, #48824 ) ) ;
#52609=CARTESIAN_POINT ( 'NONE',  ( 20.25366426268886499, -2.573118374677165754, -4.179292740214979318 ) ) ;
#52610=DIRECTION ( 'NONE',  ( -0.000000000000000000, -1.000000000000000000, -0.000000000000000000 ) ) ;
#52611=CARTESIAN_POINT ( 'NONE',  ( 17.34645602450315138, 0.4686430837609508737, 5.377443133677435760 ) ) ;
#52612=EDGE_LOOP ( 'NONE', ( #64473, #86739 ) ) ;
#52613=AXIS2_PLACEMENT_3D ( 'NONE', #106538, #114422, #46993 ) ;
#52614=DIRECTION ( 'NONE',  ( 0.000000000000000000, 0.000000000000000000, 1.000000000000000000 ) ) ;
#52615=AXIS2_PLACEMENT_3D ( 'NONE', #32439, #71688, #52061 ) ;
#52616=DIRECTION ( 'NONE',  ( 0.000000000000000000, 1.000000000000000000, 0.000000000000000000 ) ) ;
#52618=ADVANCED_FACE ( 'NONE', ( #27583 ), #107069, .T. ) ;
#52619=EDGE_CURVE ( 'NONE', #20692, #61976, #46439, .T. ) ;
#52620=EDGE_LOOP ( 'NONE', ( #78914, #116623, #23435, #112965 ) ) ;
#52621=AXIS2_PLACEMENT_3D ( 'NONE', #88715, #69068, #99189 ) ;
#52622=EDGE_LOOP ( 'NONE', ( #100416, #84944 ) ) ;
#52623=EDGE_LOOP ( 'NONE', ( #2311, #19938 ) ) ;
#52624=FACE_OUTER_BOUND ( 'NONE', #45472, .T. ) ;
#52625=CARTESIAN_POINT ( 'NONE',  ( 6.649999999999929301, 2.500000000000000000, 6.595190528383296780 ) ) ;
#52626=CARTESIAN_POINT ( 'NONE',  ( -8.350000000000013856, 2.500000000000000000, -5.802370205355744659 ) ) ;
#52627=EDGE_CURVE ( 'NONE', #76, #16047, #59002, .T. ) ;
#52628=FACE_BOUND ( 'NONE', #123614, .T. ) ;
#52629=ORIENTED_EDGE ( 'NONE', *, *, #78108, .F. ) ;
#52630=FACE_OUTER_BOUND ( 'NONE', #112537, .T. ) ;
#52631=DIRECTION ( 'NONE',  ( 0.000000000000000000, 0.000000000000000000, -1.000000000000000000 ) ) ;
#52632=VERTEX_POINT ( 'NONE', #26966 ) ;
#52633=CARTESIAN_POINT ( 'NONE',  ( 87.50000000000000000, 2.780337595463734419E-15, -7.500000000000000000 ) ) ;
#52634=DIRECTION ( 'NONE',  ( -0.000000000000000000, 1.000000000000000000, -0.000000000000000000 ) ) ;
#52635=CARTESIAN_POINT ( 'NONE',  ( -11.24999999999999822, 12.50000000000000000, 5.737276932171707422 ) ) ;
#52636=DIRECTION ( 'NONE',  ( 0.000000000000000000, 1.000000000000000000, 0.000000000000000000 ) ) ;
#52637=FACE_OUTER_BOUND ( 'NONE', #50829, .T. ) ;
#52638=LINE ( 'NONE', #90636, #86918 ) ;
#52639=FACE_OUTER_BOUND ( 'NONE', #28856, .T. ) ;
#52640=VECTOR ( 'NONE', #81565, 1000.000000000000000 ) ;
#52641=AXIS2_PLACEMENT_3D ( 'NONE', #12625, #22486, #114065 ) ;
#52642=ORIENTED_EDGE ( 'NONE', *, *, #84726, .T. ) ;
#52643=VERTEX_POINT ( 'NONE', #87157 ) ;
#52644=ORIENTED_EDGE ( 'NONE', *, *, #37721, .T. ) ;
#52645=VERTEX_POINT ( 'NONE', #96987 ) ;
#52646=CARTESIAN_POINT ( 'NONE',  ( -7.100000000000017408, 12.50000000000000000, -5.022947341949754119 ) ) ;
#52647=DIRECTION ( 'NONE',  ( 0.000000000000000000, 0.000000000000000000, -1.000000000000000000 ) ) ;
#52648=CARTESIAN_POINT ( 'NONE',  ( -2.900000000000030109, 12.50000000000000000, 0.6277270498435120194 ) ) ;
#52649=ORIENTED_EDGE ( 'NONE', *, *, #126642, .F. ) ;
#52650=FACE_BOUND ( 'NONE', #58658, .T. ) ;
#52651=AXIS2_PLACEMENT_3D ( 'NONE', #40401, #20102, #119572 ) ;
#52652=DIRECTION ( 'NONE',  ( 0.000000000000000000, 0.000000000000000000, -1.000000000000000000 ) ) ;
#52653=DIRECTION ( 'NONE',  ( 0.000000000000000000, 1.000000000000000000, 0.000000000000000000 ) ) ;
#52654=AXIS2_PLACEMENT_3D ( 'NONE', #124674, #24534, #65734 ) ;
#52655=AXIS2_PLACEMENT_3D ( 'NONE', #108747, #40692, #19065 ) ;
#52656=FACE_OUTER_BOUND ( 'NONE', #36998, .T. ) ;
#52657=EDGE_CURVE ( 'NONE', #108562, #49122, #127108, .T. ) ;
#52658=VECTOR ( 'NONE', #23940, 1000.000000000000000 ) ;
#52659=AXIS2_PLACEMENT_3D ( 'NONE', #99695, #110781, #40790 ) ;
#52660=CARTESIAN_POINT ( 'NONE',  ( 1.849999999999951017, 2.500000000000000000, -6.148780366869526226 ) ) ;
#52661=DIRECTION ( 'NONE',  ( -4.274815082592931898E-19, -0.9999939076577903929, -0.003490651415223739937 ) ) ;
#52662=LINE ( 'NONE', #112237, #95611 ) ;
#52663=FACE_OUTER_BOUND ( 'NONE', #29407, .T. ) ;
#52664=DIRECTION ( 'NONE',  ( 0.000000000000000000, 0.000000000000000000, -1.000000000000000000 ) ) ;
#52665=EDGE_CURVE ( 'NONE', #87872, #95698, #71476, .T. ) ;
#52666=FACE_OUTER_BOUND ( 'NONE', #91501, .T. ) ;
#52667=ADVANCED_FACE ( 'NONE', ( #119848 ), #12973, .T. ) ;
#52668=AXIS2_PLACEMENT_3D ( 'NONE', #99150, #79510, #38297 ) ;
#52669=ORIENTED_EDGE ( 'NONE', *, *, #89947, .F. ) ;
#52670=CONICAL_SURFACE ( 'NONE', #31754, 0.1000000000000002554, 0.003490658503988666988 ) ;
#52671=EDGE_LOOP ( 'NONE', ( #35375, #113261 ) ) ;
#52672=EDGE_LOOP ( 'NONE', ( #48197, #66264 ) ) ;
#52673=ORIENTED_EDGE ( 'NONE', *, *, #120807, .F. ) ;
#52674=EDGE_LOOP ( 'NONE', ( #111330, #41690, #27031, #55636 ) ) ;
#52675=AXIS2_PLACEMENT_3D ( 'NONE', #45962, #33564, #85855 ) ;
#52676=AXIS2_PLACEMENT_3D ( 'NONE', #113033, #114324, #24664 ) ;
#52677=EDGE_CURVE ( 'NONE', #60915, #101221, #17160, .T. ) ;
#52678=ORIENTED_EDGE ( 'NONE', *, *, #30215, .T. ) ;
#52679=FACE_OUTER_BOUND ( 'NONE', #22313, .T. ) ;
#52680=EDGE_CURVE ( 'NONE', #16531, #16470, #89745, .T. ) ;
#52681=EDGE_CURVE ( 'NONE', #122810, #122820, #6695, .T. ) ;
#52682=ORIENTED_EDGE ( 'NONE', *, *, #16829, .T. ) ;
#52683=EDGE_LOOP ( 'NONE', ( #15758, #124925, #77512, #35018 ) ) ;
#52684=AXIS2_PLACEMENT_3D ( 'NONE', #111216, #9176, #51052 ) ;
#52685=ADVANCED_FACE ( 'NONE', ( #100214 ), #79297, .T. ) ;
#52686=CONICAL_SURFACE ( 'NONE', #83970, 0.09999999999999999167, 0.003490658503988666988 ) ;
#52687=FACE_OUTER_BOUND ( 'NONE', #65070, .T. ) ;
#52688=PLANE ( 'NONE',  #14395 ) ;
#52689=LINE ( 'NONE', #69749, #25942 ) ;
#52690=ORIENTED_EDGE ( 'NONE', *, *, #101931, .T. ) ;
#52691=CARTESIAN_POINT ( 'NONE',  ( 6.049999999999932321, 2.500000000000000000, 1.818653347947321475 ) ) ;
#52692=EDGE_CURVE ( 'NONE', #60192, #118069, #40013, .T. ) ;
#52693=VERTEX_POINT ( 'NONE', #713 ) ;
#52695=DIRECTION ( 'NONE',  ( 0.000000000000000000, 0.000000000000000000, 1.000000000000000000 ) ) ;
#52696=LINE ( 'NONE', #90690, #25231 ) ;
#52697=VERTEX_POINT ( 'NONE', #51131 ) ;
#52698=EDGE_LOOP ( 'NONE', ( #34518, #100875, #61889, #46536 ) ) ;
#52699=CARTESIAN_POINT ( 'NONE',  ( -8.350000000000012079, 12.50000000000000000, 2.857883832488649301 ) ) ;
#52700=FACE_OUTER_BOUND ( 'NONE', #123427, .T. ) ;
#52701=CARTESIAN_POINT ( 'NONE',  ( 1.249999999999988454, 2.500000000000000000, -2.165063509461101710 ) ) ;
#52703=DIRECTION ( 'NONE',  ( 0.000000000000000000, -0.9999939076577903929, 0.003490651415223739937 ) ) ;
#52704=CONICAL_SURFACE ( 'NONE', #63168, 0.09999999999999999167, 0.003490658503988666988 ) ;
#52705=AXIS2_PLACEMENT_3D ( 'NONE', #72693, #75256, #53689 ) ;
#52706=DIRECTION ( 'NONE',  ( 0.000000000000000000, 1.000000000000000000, 0.000000000000000000 ) ) ;
#52707=ORIENTED_EDGE ( 'NONE', *, *, #78463, .F. ) ;
#52708=DIRECTION ( 'NONE',  ( 0.000000000000000000, 0.000000000000000000, -1.000000000000000000 ) ) ;
#52709=CONICAL_SURFACE ( 'NONE', #59070, 0.09999999999999982514, 0.003490658503988666988 ) ;
#52710=CIRCLE ( 'NONE', #123792, 0.09999999999999982514 ) ;
#52712=CARTESIAN_POINT ( 'NONE',  ( -5.000000000000022204, 2.500000000000000000, -0.6928203230275541413 ) ) ;
#52713=VECTOR ( 'NONE', #690, 1000.000000000000000 ) ;
#52714=CARTESIAN_POINT ( 'NONE',  ( -13.09999999999999254, 2.500000000000000000, 0.2464101615137777868 ) ) ;
#52715=DIRECTION ( 'NONE',  ( 0.000000000000000000, 0.000000000000000000, -1.000000000000000000 ) ) ;
#52716=AXIS2_PLACEMENT_3D ( 'NONE', #17901, #76838, #87282 ) ;
#52717=AXIS2_PLACEMENT_3D ( 'NONE', #63719, #22524, #82730 ) ;
#52718=DIRECTION ( 'NONE',  ( 0.000000000000000000, -0.9999939076577903929, 0.003490651415223739937 ) ) ;
#52719=DIRECTION ( 'NONE',  ( -0.000000000000000000, 1.000000000000000000, -0.000000000000000000 ) ) ;
#52720=VERTEX_POINT ( 'NONE', #101507 ) ;
#52721=VECTOR ( 'NONE', #99431, 1000.000000000000000 ) ;
#52722=CARTESIAN_POINT ( 'NONE',  ( 0.6499999999999566125, 2.500000000000000000, -6.741600689897077281 ) ) ;
#52723=EDGE_CURVE ( 'NONE', #33429, #66127, #65206, .T. ) ;
#52724=DIRECTION ( 'NONE',  ( -0.000000000000000000, 1.000000000000000000, -0.000000000000000000 ) ) ;
#52725=ORIENTED_EDGE ( 'NONE', *, *, #22251, .F. ) ;
#52726=ORIENTED_EDGE ( 'NONE', *, *, #114875, .T. ) ;
#52727=VERTEX_POINT ( 'NONE', #119209 ) ;
#52728=DIRECTION ( 'NONE',  ( 0.000000000000000000, 1.000000000000000000, 0.000000000000000000 ) ) ;
#52729=DIRECTION ( 'NONE',  ( 0.000000000000000000, 1.000000000000000000, 0.000000000000000000 ) ) ;
#52731=LINE ( 'NONE', #92660, #128586 ) ;
#52732=CARTESIAN_POINT ( 'NONE',  ( 4.799999999999937650, 2.500000000000000000, -0.3464101615137782364 ) ) ;
#52733=EDGE_CURVE ( 'NONE', #113918, #109879, #94555, .T. ) ;
#52734=DIRECTION ( 'NONE',  ( 0.000000000000000000, 0.000000000000000000, 1.000000000000000000 ) ) ;
#52735=LINE ( 'NONE', #92667, #115277 ) ;
#52736=CIRCLE ( 'NONE', #15154, 0.06509327318403745899 ) ;
#52737=LINE ( 'NONE', #33745, #127964 ) ;
#52738=VERTEX_POINT ( 'NONE', #40676 ) ;
#52739=CARTESIAN_POINT ( 'NONE',  ( -9.400000000000009237, 2.500000000000000000, -4.676537180435974328 ) ) ;
#52740=CARTESIAN_POINT ( 'NONE',  ( 4.349999999999940137, 2.500000000000000000, -6.941600689897078347 ) ) ;
#52741=DIRECTION ( 'NONE',  ( 0.000000000000000000, 1.000000000000000000, 0.000000000000000000 ) ) ;
#52742=DIRECTION ( 'NONE',  ( 0.000000000000000000, 0.000000000000000000, 1.000000000000000000 ) ) ;
#52743=AXIS2_PLACEMENT_3D ( 'NONE', #95923, #94624, #84808 ) ;
#52744=AXIS2_PLACEMENT_3D ( 'NONE', #40823, #32302, #110816 ) ;
#52745=ORIENTED_EDGE ( 'NONE', *, *, #71553, .F. ) ;
#52746=CARTESIAN_POINT ( 'NONE',  ( -11.25000000000000000, 12.50000000000000000, 7.122917578226811486 ) ) ;
#52747=VECTOR ( 'NONE', #116807, 1000.000000000000000 ) ;
#52748=CARTESIAN_POINT ( 'NONE',  ( -14.79999999999998472, 2.500000000000000000, 0.4464101615137758272 ) ) ;
#52749=CARTESIAN_POINT ( 'NONE',  ( -2.500000000000030642, 2.500000000000000000, -0.5928203230275541635 ) ) ;
#52750=ORIENTED_EDGE ( 'NONE', *, *, #38682, .T. ) ;
#52751=AXIS2_PLACEMENT_3D ( 'NONE', #30425, #34111, #84498 ) ;
#52752=ORIENTED_EDGE ( 'NONE', *, *, #27569, .T. ) ;
#52753=DIRECTION ( 'NONE',  ( 0.000000000000000000, 1.000000000000000000, 0.000000000000000000 ) ) ;
#52754=AXIS2_PLACEMENT_3D ( 'NONE', #91755, #3374, #14462 ) ;
#52755=ADVANCED_FACE ( 'NONE', ( #99582 ), #115368, .T. ) ;
#52756=ORIENTED_EDGE ( 'NONE', *, *, #76923, .T. ) ;
#52757=AXIS2_PLACEMENT_3D ( 'NONE', #27412, #55603, #115807 ) ;
#52758=AXIS2_PLACEMENT_3D ( 'NONE', #41299, #92307, #121131 ) ;
#52759=ORIENTED_EDGE ( 'NONE', *, *, #1074, .T. ) ;
#52760=AXIS2_PLACEMENT_3D ( 'NONE', #113365, #42060, #103563 ) ;
#52761=DIRECTION ( 'NONE',  ( 0.000000000000000000, -0.9999939076577903929, 0.003490651415223739937 ) ) ;
#52763=LINE ( 'NONE', #54674, #30046 ) ;
#52764=LINE ( 'NONE', #120862, #92274 ) ;
#52765=CARTESIAN_POINT ( 'NONE',  ( -8.950000000000008171, 2.500000000000000000, -2.611473670974877592 ) ) ;
#52766=EDGE_CURVE ( 'NONE', #39661, #78151, #88182, .T. ) ;
#52767=VERTEX_POINT ( 'NONE', #81224 ) ;
#52768=CIRCLE ( 'NONE', #50718, 0.06509327318403743123 ) ;
#52769=DIRECTION ( 'NONE',  ( -0.000000000000000000, 1.000000000000000000, -0.000000000000000000 ) ) ;
#52770=LINE ( 'NONE', #60202, #95888 ) ;
#52771=ORIENTED_EDGE ( 'NONE', *, *, #86537, .T. ) ;
#52772=EDGE_CURVE ( 'NONE', #121359, #69185, #102150, .T. ) ;
#52773=DIRECTION ( 'NONE',  ( -0.000000000000000000, 1.000000000000000000, -0.000000000000000000 ) ) ;
#52774=CARTESIAN_POINT ( 'NONE',  ( 17.49862860983209600, -2.500000000000000000, 4.081131818001135336 ) ) ;
#52775=EDGE_CURVE ( 'NONE', #96170, #109430, #100807, .T. ) ;
#52776=ORIENTED_EDGE ( 'NONE', *, *, #10641, .F. ) ;
#52777=ORIENTED_EDGE ( 'NONE', *, *, #98044, .T. ) ;
#52778=EDGE_CURVE ( 'NONE', #12245, #125864, #79896, .T. ) ;
#52779=ORIENTED_EDGE ( 'NONE', *, *, #125847, .T. ) ;
#52780=VERTEX_POINT ( 'NONE', #21656 ) ;
#52781=DIRECTION ( 'NONE',  ( 0.000000000000000000, -0.000000000000000000, 1.000000000000000000 ) ) ;
#52782=CARTESIAN_POINT ( 'NONE',  ( 14.93723468939127841, 2.500000000000000000, 6.174425106950392816 ) ) ;
#52783=DIRECTION ( 'NONE',  ( 0.000000000000000000, 0.000000000000000000, -1.000000000000000000 ) ) ;
#52784=AXIS2_PLACEMENT_3D ( 'NONE', #79323, #128430, #9275 ) ;
#52785=EDGE_CURVE ( 'NONE', #86677, #46102, #111262, .T. ) ;
#52786=FACE_BOUND ( 'NONE', #102993, .T. ) ;
#52787=ORIENTED_EDGE ( 'NONE', *, *, #75858, .T. ) ;
#52789=CARTESIAN_POINT ( 'NONE',  ( 7.299999999999924327, 2.500000000000000000, 0.3464101615137735735 ) ) ;
#52790=CARTESIAN_POINT ( 'NONE',  ( -9.400000000000007461, 12.50000000000000000, 3.983716857408420076 ) ) ;
#52791=VECTOR ( 'NONE', #102397, 1000.000000000000000 ) ;
#52792=CIRCLE ( 'NONE', #105104, 0.06509327318403745899 ) ;
#52793=CARTESIAN_POINT ( 'NONE',  ( -1.250000000000037970, 2.500000000000000000, 7.188010851410848723 ) ) ;
#52794=AXIS2_PLACEMENT_3D ( 'NONE', #3625, #121452, #92007 ) ;
#52795=DIRECTION ( 'NONE',  ( 0.000000000000000000, 0.000000000000000000, -1.000000000000000000 ) ) ;
#52796=DIRECTION ( 'NONE',  ( 0.000000000000000000, -0.000000000000000000, 1.000000000000000000 ) ) ;
#52797=CIRCLE ( 'NONE', #117523, 0.1000000000000000056 ) ;
#52798=CONICAL_SURFACE ( 'NONE', #121752, 0.09999999999999982514, 0.003490658503988666988 ) ;
#52799=DIRECTION ( 'NONE',  ( 0.000000000000000000, 0.000000000000000000, 1.000000000000000000 ) ) ;
#52800=CIRCLE ( 'NONE', #42454, 0.1000000000000002554 ) ;
#52801=EDGE_LOOP ( 'NONE', ( #74048, #96560, #3269, #82906 ) ) ;
#52802=EDGE_LOOP ( 'NONE', ( #32722, #82457 ) ) ;
#52803=ORIENTED_EDGE ( 'NONE', *, *, #53272, .T. ) ;
#52804=ORIENTED_EDGE ( 'NONE', *, *, #102954, .F. ) ;
#52805=AXIS2_PLACEMENT_3D ( 'NONE', #75855, #93109, #13878 ) ;
#52806=VERTEX_POINT ( 'NONE', #91680 ) ;
#52807=DIRECTION ( 'NONE',  ( 0.000000000000000000, 0.000000000000000000, -1.000000000000000000 ) ) ;
#52808=AXIS2_PLACEMENT_3D ( 'NONE', #5832, #45148, #106623 ) ;
#52809=DIRECTION ( 'NONE',  ( 0.000000000000000000, -0.9999939076577903929, 0.003490651415223739937 ) ) ;
#52810=VERTEX_POINT ( 'NONE', #111976 ) ;
#52811=FACE_BOUND ( 'NONE', #77148, .T. ) ;
#52812=AXIS2_PLACEMENT_3D ( 'NONE', #58692, #78346, #38426 ) ;
#52813=DIRECTION ( 'NONE',  ( 0.000000000000000000, 1.000000000000000000, 0.000000000000000000 ) ) ;
#52814=ADVANCED_FACE ( 'NONE', ( #50458 ), #86129, .T. ) ;
#52815=EDGE_LOOP ( 'NONE', ( #94754, #57225 ) ) ;
#52816=DIRECTION ( 'NONE',  ( -0.000000000000000000, 1.000000000000000000, -0.000000000000000000 ) ) ;
#52817=DIRECTION ( 'NONE',  ( -0.000000000000000000, 1.000000000000000000, -0.000000000000000000 ) ) ;
#52818=DIRECTION ( 'NONE',  ( 0.000000000000000000, 1.000000000000000000, 0.000000000000000000 ) ) ;
#52819=EDGE_LOOP ( 'NONE', ( #30348, #54399, #112334, #48025 ) ) ;
#52820=CARTESIAN_POINT ( 'NONE',  ( -0.8500000000000382805, 12.50000000000000000, -5.802370205355749988 ) ) ;
#52821=ADVANCED_FACE ( 'NONE', ( #62236 ), #2510, .T. ) ;
#52822=CONICAL_SURFACE ( 'NONE', #86257, 0.1000000000000000472, 0.003490658503988666988 ) ;
#52823=ORIENTED_EDGE ( 'NONE', *, *, #14959, .T. ) ;
#52824=VERTEX_POINT ( 'NONE', #123690 ) ;
#52825=ORIENTED_EDGE ( 'NONE', *, *, #109163, .F. ) ;
#52826=ADVANCED_FACE ( 'NONE', ( #4548 ), #92406, .T. ) ;
#52827=CARTESIAN_POINT ( 'NONE',  ( -3.749999999999994671, 12.50000000000000000, -6.560283801567339701 ) ) ;
#52828=FACE_OUTER_BOUND ( 'NONE', #9660, .T. ) ;
#52829=CARTESIAN_POINT ( 'NONE',  ( -7.100000000000018296, 2.500000000000000000, -4.230127018922201998 ) ) ;
#52830=ADVANCED_FACE ( 'NONE', ( #32787 ), #77833, .T. ) ;
#52831=ORIENTED_EDGE ( 'NONE', *, *, #65352, .T. ) ;
#52832=CARTESIAN_POINT ( 'NONE',  ( -13.54999999999999005, 2.500000000000000000, 2.511473670974877503 ) ) ;
#52833=EDGE_CURVE ( 'NONE', #72795, #30951, #21399, .T. ) ;
#52834=CIRCLE ( 'NONE', #71705, 0.1000000000000002554 ) ;
#52835=AXIS2_PLACEMENT_3D ( 'NONE', #16071, #105106, #95944 ) ;
#52836=CIRCLE ( 'NONE', #71611, 0.09999999999999982514 ) ;
#52837=DIRECTION ( 'NONE',  ( 0.6795087154616719083, 3.181775308912716821E-15, 0.7336674352945131705 ) ) ;
#52838=CARTESIAN_POINT ( 'NONE',  ( -4.350000000000023626, 2.500000000000000000, -1.818653347947325916 ) ) ;
#52839=EDGE_CURVE ( 'NONE', #2439, #53221, #90341, .T. ) ;
#52841=EDGE_LOOP ( 'NONE', ( #16376, #23335, #86768, #116227 ) ) ;
#52842=DIRECTION ( 'NONE',  ( 0.000000000000000000, 0.000000000000000000, 1.000000000000000000 ) ) ;
#52843=CONICAL_SURFACE ( 'NONE', #100950, 0.09999999999999982514, 0.003490658503988666988 ) ;
#52844=VERTEX_POINT ( 'NONE', #73973 ) ;
#52845=FACE_OUTER_BOUND ( 'NONE', #367, .T. ) ;
#52846=EDGE_CURVE ( 'NONE', #126729, #114539, #33927, .T. ) ;
#52847=VECTOR ( 'NONE', #86473, 1000.000000000000000 ) ;
#52848=EDGE_CURVE ( 'NONE', #112012, #37787, #98759, .T. ) ;
#52849=VERTEX_POINT ( 'NONE', #65431 ) ;
#52850=CIRCLE ( 'NONE', #38282, 0.09999999999999982514 ) ;
#52851=ORIENTED_EDGE ( 'NONE', *, *, #13191, .F. ) ;
#52853=DIRECTION ( 'NONE',  ( 0.000000000000000000, -0.000000000000000000, 1.000000000000000000 ) ) ;
#52854=CARTESIAN_POINT ( 'NONE',  ( -1.850000000000033396, 12.50000000000000000, -6.841600689897077814 ) ) ;
#52855=FACE_OUTER_BOUND ( 'NONE', #15679, .T. ) ;
#52857=AXIS2_PLACEMENT_3D ( 'NONE', #112526, #62141, #24141 ) ;
#52859=ORIENTED_EDGE ( 'NONE', *, *, #50474, .T. ) ;
#52860=VECTOR ( 'NONE', #127660, 1000.000000000000000 ) ;
#52861=CARTESIAN_POINT ( 'NONE',  ( 0.5999999999999547917, 12.50000000000000000, 3.983716857408420076 ) ) ;
#52862=DIRECTION ( 'NONE',  ( 0.000000000000000000, -0.000000000000000000, 1.000000000000000000 ) ) ;
#52863=AXIS2_PLACEMENT_3D ( 'NONE', #79753, #98735, #9077 ) ;
#52864=AXIS2_PLACEMENT_3D ( 'NONE', #71714, #22635, #111647 ) ;
#52866=DIRECTION ( 'NONE',  ( -0.000000000000000000, 1.000000000000000000, -0.000000000000000000 ) ) ;
#52867=EDGE_LOOP ( 'NONE', ( #6020, #39383, #120685, #47913 ) ) ;
#52868=ORIENTED_EDGE ( 'NONE', *, *, #77508, .T. ) ;
#52869=DIRECTION ( 'NONE',  ( 0.000000000000000000, 1.000000000000000000, 0.000000000000000000 ) ) ;
#52870=CIRCLE ( 'NONE', #128180, 0.09999999999999982514 ) ;
#52871=ORIENTED_EDGE ( 'NONE', *, *, #61301, .F. ) ;
#52872=CARTESIAN_POINT ( 'NONE',  ( 7.899999999999924860, 2.500000000000000000, 5.122947341949749323 ) ) ;
#52873=CARTESIAN_POINT ( 'NONE',  ( 0.6499999999999561684, 12.50000000000000000, -1.818653347947325916 ) ) ;
#52874=CARTESIAN_POINT ( 'NONE',  ( 1.649999999999951950, 2.500000000000000000, -7.188010851410854052 ) ) ;
#52875=ORIENTED_EDGE ( 'NONE', *, *, #107637, .T. ) ;
#52876=VECTOR ( 'NONE', #20152, 1000.000000000000000 ) ;
#52877=CARTESIAN_POINT ( 'NONE',  ( 7.099999999999928590, 12.50000000000000000, -4.265033745738164406 ) ) ;
#52878=CARTESIAN_POINT ( 'NONE',  ( 9.149999999999916866, 2.500000000000000000, -1.472243186433550122 ) ) ;
#52879=CARTESIAN_POINT ( 'NONE',  ( -3.150000000000033218, 2.500000000000000000, -6.941600689897078347 ) ) ;
#52880=CARTESIAN_POINT ( 'NONE',  ( -14.34999999999998543, 12.50000000000000000, 1.753560074763288013 ) ) ;
#52881=FACE_OUTER_BOUND ( 'NONE', #99700, .T. ) ;
#52882=EDGE_LOOP ( 'NONE', ( #51993, #77858, #50600, #31685 ) ) ;
#52883=CARTESIAN_POINT ( 'NONE',  ( 10.19999999999991047, 2.500000000000000000, -3.883716857408426648 ) ) ;
#52884=EDGE_CURVE ( 'NONE', #20798, #60736, #111355, .T. ) ;
#52885=CARTESIAN_POINT ( 'NONE',  ( 32.28071041560937715, -1.401423001991335182, 4.680142630335650367 ) ) ;
#52886=ORIENTED_EDGE ( 'NONE', *, *, #126095, .T. ) ;
#52887=ORIENTED_EDGE ( 'NONE', *, *, #45132, .T. ) ;
#52888=AXIS2_PLACEMENT_3D ( 'NONE', #73334, #74633, #114545 ) ;
#52890=DIRECTION ( 'NONE',  ( 0.000000000000000000, -0.000000000000000000, 1.000000000000000000 ) ) ;
#52891=DIRECTION ( 'NONE',  ( -0.000000000000000000, 1.000000000000000000, -0.000000000000000000 ) ) ;
#52892=CARTESIAN_POINT ( 'NONE',  ( 11.64999999999990443, 2.500000000000000000, 2.857883832488649301 ) ) ;
#52893=FACE_OUTER_BOUND ( 'NONE', #64491, .T. ) ;
#52894=EDGE_CURVE ( 'NONE', #26891, #112496, #96692, .T. ) ;
#52895=CIRCLE ( 'NONE', #86320, 0.1000000000000002554 ) ;
#52896=CARTESIAN_POINT ( 'NONE',  ( -3.550000000000030909, 12.50000000000000000, -6.776507416713040577 ) ) ;
#52897=DIRECTION ( 'NONE',  ( 0.000000000000000000, 0.000000000000000000, 1.000000000000000000 ) ) ;
#52898=AXIS2_PLACEMENT_3D ( 'NONE', #60860, #60241, #81772 ) ;
#52899=PLANE ( 'NONE',  #40687 ) ;
#52900=CARTESIAN_POINT ( 'NONE',  ( 5.399999999999932854, 2.500000000000000000, 3.537306695894645081 ) ) ;
#52901=CONICAL_SURFACE ( 'NONE', #17359, 0.1000000000000002554, 0.003490658503988666988 ) ;
#52902=AXIS2_PLACEMENT_3D ( 'NONE', #112936, #91358, #31807 ) ;
#52903=CARTESIAN_POINT ( 'NONE',  ( 3.299999999999944755, 2.500000000000000000, -2.385244779468109755E-15 ) ) ;
#52905=AXIS2_PLACEMENT_3D ( 'NONE', #26805, #98752, #56878 ) ;
#52906=ORIENTED_EDGE ( 'NONE', *, *, #29059, .F. ) ;
#52907=CONICAL_SURFACE ( 'NONE', #109326, 0.1000000000000002554, 0.003490658503988666988 ) ;
#52908=ORIENTED_EDGE ( 'NONE', *, *, #85329, .F. ) ;
#52909=CIRCLE ( 'NONE', #126047, 0.06509327318403745899 ) ;
#52910=AXIS2_PLACEMENT_3D ( 'NONE', #120959, #31316, #12282 ) ;
#52911=EDGE_LOOP ( 'NONE', ( #113912, #81330 ) ) ;
#52912=FACE_OUTER_BOUND ( 'NONE', #49814, .T. ) ;
#52913=DIRECTION ( 'NONE',  ( 0.000000000000000000, 0.000000000000000000, 1.000000000000000000 ) ) ;
#52914=AXIS2_PLACEMENT_3D ( 'NONE', #69466, #60942, #108748 ) ;
#52915=ORIENTED_EDGE ( 'NONE', *, *, #30978, .F. ) ;
#52916=DIRECTION ( 'NONE',  ( 0.000000000000000000, 1.000000000000000000, 0.000000000000000000 ) ) ;
#52917=DIRECTION ( 'NONE',  ( -0.000000000000000000, -1.000000000000000000, -0.000000000000000000 ) ) ;
#52918=CARTESIAN_POINT ( 'NONE',  ( -11.64999999999999680, 2.500000000000000000, 2.065063509461097624 ) ) ;
#52919=VERTEX_POINT ( 'NONE', #104082 ) ;
#52920=DIRECTION ( 'NONE',  ( -0.000000000000000000, 1.000000000000000000, -0.000000000000000000 ) ) ;
#52921=AXIS2_PLACEMENT_3D ( 'NONE', #86579, #115371, #8016 ) ;
#52922=PLANE ( 'NONE',  #102285 ) ;
#52923=ORIENTED_EDGE ( 'NONE', *, *, #44218, .T. ) ;
#52924=ORIENTED_EDGE ( 'NONE', *, *, #68032, .F. ) ;
#52925=ORIENTED_EDGE ( 'NONE', *, *, #104485, .T. ) ;
#52926=ORIENTED_EDGE ( 'NONE', *, *, #107088, .F. ) ;
#52927=CARTESIAN_POINT ( 'NONE',  ( 12.89999999999990088, 2.500000000000000000, 4.330127018922196314 ) ) ;
#52928=DIRECTION ( 'NONE',  ( 0.000000000000000000, 0.000000000000000000, 1.000000000000000000 ) ) ;
#52929=CARTESIAN_POINT ( 'NONE',  ( 6.849999999999929479, 12.50000000000000000, 6.083687093685482772 ) ) ;
#52930=CIRCLE ( 'NONE', #111503, 0.1000000000000002554 ) ;
#52931=FACE_OUTER_BOUND ( 'NONE', #107562, .T. ) ;
#52932=EDGE_CURVE ( 'NONE', #106610, #65076, #128015, .T. ) ;
#52933=AXIS2_PLACEMENT_3D ( 'NONE', #85176, #14479, #115923 ) ;
#52934=EDGE_LOOP ( 'NONE', ( #55623, #3377 ) ) ;
#52935=DIRECTION ( 'NONE',  ( -4.274815082592931898E-19, -0.9999939076577903929, -0.003490651415223739937 ) ) ;
#52936=ORIENTED_EDGE ( 'NONE', *, *, #60767, .F. ) ;
#52937=CARTESIAN_POINT ( 'NONE',  ( -3.350000000000028511, 12.50000000000000000, -1.472243186433550122 ) ) ;
#52938=CARTESIAN_POINT ( 'NONE',  ( 7.306656945292925975, -2.500000000000506706, -9.704971168059893571 ) ) ;
#52939=EDGE_CURVE ( 'NONE', #126753, #103801, #50749, .T. ) ;
#52940=DIRECTION ( 'NONE',  ( 0.000000000000000000, 0.000000000000000000, 1.000000000000000000 ) ) ;
#52941=PLANE ( 'NONE',  #38085 ) ;
#52942=AXIS2_PLACEMENT_3D ( 'NONE', #22871, #63422, #2542 ) ;
#52943=EDGE_CURVE ( 'NONE', #29223, #54633, #36076, .T. ) ;
#52944=CIRCLE ( 'NONE', #13211, 0.1000000000000002554 ) ;
#52945=AXIS2_PLACEMENT_3D ( 'NONE', #45614, #55423, #85521 ) ;
#52946=ORIENTED_EDGE ( 'NONE', *, *, #100693, .F. ) ;
#52948=ORIENTED_EDGE ( 'NONE', *, *, #11316, .F. ) ;
#52949=EDGE_CURVE ( 'NONE', #56299, #102282, #56982, .T. ) ;
#52950=EDGE_CURVE ( 'NONE', #87296, #112974, #84436, .T. ) ;
#52951=EDGE_LOOP ( 'NONE', ( #5434, #88004, #124589, #90970 ) ) ;
#52952=FACE_OUTER_BOUND ( 'NONE', #125605, .T. ) ;
#52953=CARTESIAN_POINT ( 'NONE',  ( -12.89999999999999147, 2.500000000000000000, 0.1000000000000018513 ) ) ;
#52954=DIRECTION ( 'NONE',  ( -0.000000000000000000, -1.000000000000000000, -0.000000000000000000 ) ) ;
#52955=EDGE_CURVE ( 'NONE', #30530, #114894, #63518, .T. ) ;
#52956=FACE_BOUND ( 'NONE', #56899, .T. ) ;
#52957=DIRECTION ( 'NONE',  ( 0.000000000000000000, 0.000000000000000000, 1.000000000000000000 ) ) ;
#52958=CARTESIAN_POINT ( 'NONE',  ( 12.49999999999990408, 2.500000000000000000, -3.637306695894650055 ) ) ;
#52959=CARTESIAN_POINT ( 'NONE',  ( -9.350000000000004974, 2.500000000000000000, 6.941600689897073018 ) ) ;
#52960=AXIS2_PLACEMENT_3D ( 'NONE', #98426, #59845, #68982 ) ;
#52963=AXIS2_PLACEMENT_3D ( 'NONE', #17375, #66487, #4324 ) ;
#52964=DIRECTION ( 'NONE',  ( 0.000000000000000000, 1.000000000000000000, 0.000000000000000000 ) ) ;
#52965=EDGE_LOOP ( 'NONE', ( #14727, #29996, #76676, #89538 ) ) ;
#52966=DIRECTION ( 'NONE',  ( 0.000000000000000000, 1.000000000000000000, 0.000000000000000000 ) ) ;
#52967=ORIENTED_EDGE ( 'NONE', *, *, #66364, .T. ) ;
#52968=ORIENTED_EDGE ( 'NONE', *, *, #64482, .F. ) ;
#52969=FACE_OUTER_BOUND ( 'NONE', #103735, .T. ) ;
#52970=DIRECTION ( 'NONE',  ( 0.000000000000000000, 0.000000000000000000, -1.000000000000000000 ) ) ;
#52971=FACE_BOUND ( 'NONE', #20108, .T. ) ;
#52972=DIRECTION ( 'NONE',  ( -0.000000000000000000, -1.000000000000000000, -0.000000000000000000 ) ) ;
#52973=AXIS2_PLACEMENT_3D ( 'NONE', #15004, #25485, #124990 ) ;
#52974=ORIENTED_EDGE ( 'NONE', *, *, #98971, .F. ) ;
#52975=LINE ( 'NONE', #83729, #82231 ) ;
#52976=AXIS2_PLACEMENT_3D ( 'NONE', #31355, #111160, #101373 ) ;
#52977=DIRECTION ( 'NONE',  ( -4.274815082592931898E-19, -0.9999939076577903929, -0.003490651415223739937 ) ) ;
#52978=ORIENTED_EDGE ( 'NONE', *, *, #117003, .T. ) ;
#52979=DIRECTION ( 'NONE',  ( 0.000000000000000000, 1.000000000000000000, 0.000000000000000000 ) ) ;
#52980=PLANE ( 'NONE',  #32415 ) ;
#52981=CIRCLE ( 'NONE', #2804, 0.1000000000000002554 ) ;
#52982=CONICAL_SURFACE ( 'NONE', #11204, 0.1000000000000000472, 0.003490658503988666988 ) ;
#52983=AXIS2_PLACEMENT_3D ( 'NONE', #98679, #68583, #118979 ) ;
#52984=EDGE_CURVE ( 'NONE', #66538, #105977, #73317, .T. ) ;
#52985=ORIENTED_EDGE ( 'NONE', *, *, #124170, .F. ) ;
#52986=EDGE_CURVE ( 'NONE', #117024, #123082, #54938, .T. ) ;
#52987=DIRECTION ( 'NONE',  ( -4.274815082592931898E-19, -0.9999939076577903929, -0.003490651415223739937 ) ) ;
#52988=DIRECTION ( 'NONE',  ( 0.000000000000000000, 0.000000000000000000, 1.000000000000000000 ) ) ;
#52989=EDGE_CURVE ( 'NONE', #67694, #97521, #24875, .T. ) ;
#52990=CONICAL_SURFACE ( 'NONE', #67648, 0.09999999999999982514, 0.003490658503988666988 ) ;
#52991=ORIENTED_EDGE ( 'NONE', *, *, #36264, .T. ) ;
#52992=CONICAL_SURFACE ( 'NONE', #25804, 0.1000000000000000472, 0.003490658503988666988 ) ;
#52993=DIRECTION ( 'NONE',  ( -0.000000000000000000, 1.000000000000000000, -0.000000000000000000 ) ) ;
#52994=DIRECTION ( 'NONE',  ( -0.000000000000000000, 1.000000000000000000, -0.000000000000000000 ) ) ;
#52995=LINE ( 'NONE', #81167, #78623 ) ;
#52996=AXIS2_PLACEMENT_3D ( 'NONE', #29214, #118859, #119496 ) ;
#52997=EDGE_CURVE ( 'NONE', #87479, #43021, #69507, .T. ) ;
#52998=AXIS2_PLACEMENT_3D ( 'NONE', #14548, #25033, #114062 ) ;
#52999=ORIENTED_EDGE ( 'NONE', *, *, #77810, .F. ) ;
#53000=ORIENTED_EDGE ( 'NONE', *, *, #68882, .F. ) ;
#53001=EDGE_CURVE ( 'NONE', #123441, #18337, #45169, .T. ) ;
#53003=EDGE_CURVE ( 'NONE', #88166, #129005, #71578, .T. ) ;
#53004=ORIENTED_EDGE ( 'NONE', *, *, #65149, .F. ) ;
#53005=LINE ( 'NONE', #13045, #97173 ) ;
#53006=DIRECTION ( 'NONE',  ( 0.000000000000000000, 1.000000000000000000, 0.000000000000000000 ) ) ;
#53007=EDGE_CURVE ( 'NONE', #66455, #6359, #88280, .T. ) ;
#53008=EDGE_CURVE ( 'NONE', #82164, #53598, #8864, .T. ) ;
#53009=VERTEX_POINT ( 'NONE', #26809 ) ;
#53010=DIRECTION ( 'NONE',  ( 0.000000000000000000, 0.000000000000000000, -1.000000000000000000 ) ) ;
#53011=CARTESIAN_POINT ( 'NONE',  ( -0.4000000000000339950, 2.500000000000000000, 0.5928203230275517210 ) ) ;
#53012=DIRECTION ( 'NONE',  ( 0.000000000000000000, 1.000000000000000000, 0.000000000000000000 ) ) ;
#53013=DIRECTION ( 'NONE',  ( 0.000000000000000000, 0.000000000000000000, 1.000000000000000000 ) ) ;
#53014=DIRECTION ( 'NONE',  ( -4.274815082592931898E-19, -0.9999939076577903929, -0.003490651415223739937 ) ) ;
#53015=EDGE_CURVE ( 'NONE', #22721, #98931, #31876, .T. ) ;
#53016=VECTOR ( 'NONE', #113962, 1000.000000000000000 ) ;
#53017=VERTEX_POINT ( 'NONE', #40345 ) ;
#53018=ORIENTED_EDGE ( 'NONE', *, *, #86026, .T. ) ;
#53019=DIRECTION ( 'NONE',  ( 0.000000000000000000, 1.000000000000000000, 0.000000000000000000 ) ) ;
#53020=ORIENTED_EDGE ( 'NONE', *, *, #15968, .F. ) ;
#53021=CARTESIAN_POINT ( 'NONE',  ( -11.44999999999999929, 2.500000000000000000, -6.248780366869523206 ) ) ;
#53022=VERTEX_POINT ( 'NONE', #107940 ) ;
#53023=ORIENTED_EDGE ( 'NONE', *, *, #74553, .T. ) ;
#53024=ORIENTED_EDGE ( 'NONE', *, *, #84045, .T. ) ;
#53025=CARTESIAN_POINT ( 'NONE',  ( -4.800000000000026468, 2.500000000000000000, -4.676537180435978769 ) ) ;
#53026=AXIS2_PLACEMENT_3D ( 'NONE', #105241, #15561, #95432 ) ;
#53027=VECTOR ( 'NONE', #47345, 1000.000000000000000 ) ;
#53028=DIRECTION ( 'NONE',  ( 0.000000000000000000, 0.000000000000000000, 1.000000000000000000 ) ) ;
#53029=AXIS2_PLACEMENT_3D ( 'NONE', #73694, #14127, #95286 ) ;
#53030=DIRECTION ( 'NONE',  ( -0.000000000000000000, -1.000000000000000000, -0.000000000000000000 ) ) ;
#53031=FACE_OUTER_BOUND ( 'NONE', #114333, .T. ) ;
#53032=CARTESIAN_POINT ( 'NONE',  ( 9.149999999999920419, 2.500000000000000000, -7.088010851410853519 ) ) ;
#53033=PLANE ( 'NONE',  #33989 ) ;
#53034=CARTESIAN_POINT ( 'NONE',  ( 12.89999999999990266, 2.500000000000000000, -5.122947341949753763 ) ) ;
#53035=CARTESIAN_POINT ( 'NONE',  ( 7.899999999999924860, 12.50000000000000000, -3.637306695894650055 ) ) ;
#53036=EDGE_CURVE ( 'NONE', #112593, #11592, #7801, .T. ) ;
#53037=AXIS2_PLACEMENT_3D ( 'NONE', #58759, #129460, #78419 ) ;
#53038=AXIS2_PLACEMENT_3D ( 'NONE', #12140, #92650, #120820 ) ;
#53040=CIRCLE ( 'NONE', #94890, 0.09999999999999999167 ) ;
#53041=EDGE_LOOP ( 'NONE', ( #125787, #58248 ) ) ;
#53042=AXIS2_PLACEMENT_3D ( 'NONE', #84476, #94945, #29268 ) ;
#53043=DIRECTION ( 'NONE',  ( 0.000000000000000000, 1.000000000000000000, 0.000000000000000000 ) ) ;
#53044=ORIENTED_EDGE ( 'NONE', *, *, #64285, .F. ) ;
#53045=ORIENTED_EDGE ( 'NONE', *, *, #28759, .F. ) ;
#53046=CARTESIAN_POINT ( 'NONE',  ( -13.74999999999995381, 12.50000000000000000, -2.099970236277062252 ) ) ;
#53047=DIRECTION ( 'NONE',  ( -0.000000000000000000, -1.000000000000000000, -0.000000000000000000 ) ) ;
#53048=FACE_OUTER_BOUND ( 'NONE', #15311, .T. ) ;
#53049=FACE_OUTER_BOUND ( 'NONE', #12664, .T. ) ;
#53050=EDGE_CURVE ( 'NONE', #95287, #67756, #121745, .T. ) ;
#53051=DIRECTION ( 'NONE',  ( 0.000000000000000000, 0.000000000000000000, -1.000000000000000000 ) ) ;
#53052=AXIS2_PLACEMENT_3D ( 'NONE', #6077, #96395, #46672 ) ;
#53053=PLANE ( 'NONE',  #40948 ) ;
#53054=AXIS2_PLACEMENT_3D ( 'NONE', #60481, #92487, #50633 ) ;
#53055=AXIS2_PLACEMENT_3D ( 'NONE', #114342, #123511, #15488 ) ;
#53056=DIRECTION ( 'NONE',  ( -0.000000000000000000, -1.000000000000000000, -0.000000000000000000 ) ) ;
#53057=VERTEX_POINT ( 'NONE', #66716 ) ;
#53058=CIRCLE ( 'NONE', #111535, 0.09999999999999982514 ) ;
#53059=AXIS2_PLACEMENT_3D ( 'NONE', #57801, #98344, #56490 ) ;
#53060=EDGE_LOOP ( 'NONE', ( #72968, #104951, #47023, #29153 ) ) ;
#53061=ORIENTED_EDGE ( 'NONE', *, *, #34029, .F. ) ;
#53062=ORIENTED_EDGE ( 'NONE', *, *, #91397, .F. ) ;
#53063=ORIENTED_EDGE ( 'NONE', *, *, #7885, .F. ) ;
#53064=DIRECTION ( 'NONE',  ( -0.000000000000000000, -1.000000000000000000, -0.000000000000000000 ) ) ;
#53065=DIRECTION ( 'NONE',  ( 0.000000000000000000, -0.9999939076577903929, 0.003490651415223739937 ) ) ;
#53066=CARTESIAN_POINT ( 'NONE',  ( 0.6499999999999543920, 12.50000000000000000, 6.083687093685483660 ) ) ;
#53067=CARTESIAN_POINT ( 'NONE',  ( -0.8500000000000395017, 12.50000000000000000, 2.165063509461097713 ) ) ;
#53068=FACE_OUTER_BOUND ( 'NONE', #50676, .T. ) ;
#53069=ORIENTED_EDGE ( 'NONE', *, *, #3017, .T. ) ;
#53070=DIRECTION ( 'NONE',  ( -0.000000000000000000, -1.000000000000000000, -0.000000000000000000 ) ) ;
#53071=AXIS2_PLACEMENT_3D ( 'NONE', #14848, #66547, #125475 ) ;
#53072=CIRCLE ( 'NONE', #76057, 0.1000000000000002554 ) ;
#53073=DIRECTION ( 'NONE',  ( -0.000000000000000000, 1.000000000000000000, -0.000000000000000000 ) ) ;
#53074=FACE_OUTER_BOUND ( 'NONE', #72901, .T. ) ;
#53075=CARTESIAN_POINT ( 'NONE',  ( 10.84999999999990905, 12.50000000000000000, 2.857883832488649301 ) ) ;
#53076=VERTEX_POINT ( 'NONE', #18269 ) ;
#53077=AXIS2_PLACEMENT_3D ( 'NONE', #79619, #21337, #41657 ) ;
#53078=CIRCLE ( 'NONE', #843, 0.06509327318403745899 ) ;
#53079=ORIENTED_EDGE ( 'NONE', *, *, #54680, .F. ) ;
#53080=ORIENTED_EDGE ( 'NONE', *, *, #126696, .F. ) ;
#53081=AXIS2_PLACEMENT_3D ( 'NONE', #121158, #62252, #122461 ) ;
#53082=DIRECTION ( 'NONE',  ( 0.000000000000000000, 1.000000000000000000, 0.000000000000000000 ) ) ;
#53083=CARTESIAN_POINT ( 'NONE',  ( 1.649999999999950617, 2.500000000000000000, 2.265063509461097357 ) ) ;
#53085=VECTOR ( 'NONE', #3821, 1000.000000000000000 ) ;
#53086=AXIS2_PLACEMENT_3D ( 'NONE', #27560, #124510, #106773 ) ;
#53087=AXIS2_PLACEMENT_3D ( 'NONE', #46054, #85945, #57149 ) ;
#53088=EDGE_CURVE ( 'NONE', #99498, #96622, #65301, .T. ) ;
#53089=AXIS2_PLACEMENT_3D ( 'NONE', #29542, #61598, #69450 ) ;
#53090=VERTEX_POINT ( 'NONE', #56880 ) ;
#53091=CARTESIAN_POINT ( 'NONE',  ( 2.499999999999947153, 12.50000000000000000, 3.637306695894644726 ) ) ;
#53092=DIRECTION ( 'NONE',  ( 0.000000000000000000, 1.000000000000000000, 0.000000000000000000 ) ) ;
#53093=CARTESIAN_POINT ( 'NONE',  ( 5.449999999999934452, 12.50000000000000000, 2.165063509461097713 ) ) ;
#53094=CARTESIAN_POINT ( 'NONE',  ( -7.100000000000013856, 12.50000000000000000, 3.637306695894644726 ) ) ;
#53095=ADVANCED_FACE ( 'NONE', ( #99902 ), #82036, .T. ) ;
#53096=DIRECTION ( 'NONE',  ( 0.000000000000000000, 0.000000000000000000, 1.000000000000000000 ) ) ;
#53097=ORIENTED_EDGE ( 'NONE', *, *, #111799, .F. ) ;
#53098=ADVANCED_FACE ( 'NONE', ( #35982 ), #77920, .T. ) ;
#53099=ADVANCED_FACE ( 'NONE', ( #116461 ), #34020, .T. ) ;
#53100=ORIENTED_EDGE ( 'NONE', *, *, #85889, .T. ) ;
#53101=EDGE_CURVE ( 'NONE', #53201, #53951, #61214, .T. ) ;
#53102=DIRECTION ( 'NONE',  ( 0.000000000000000000, -0.9999939076577903929, 0.003490651415223739937 ) ) ;
#53103=EDGE_CURVE ( 'NONE', #125340, #95314, #77198, .T. ) ;
#53105=DIRECTION ( 'NONE',  ( 0.000000000000000000, 1.000000000000000000, 0.000000000000000000 ) ) ;
#53106=DIRECTION ( 'NONE',  ( -0.000000000000000000, 1.000000000000000000, -0.000000000000000000 ) ) ;
#53107=CONICAL_SURFACE ( 'NONE', #126263, 0.1000000000000002554, 0.003490658503988666988 ) ;
#53108=DIRECTION ( 'NONE',  ( -0.000000000000000000, -1.000000000000000000, -0.000000000000000000 ) ) ;
#53109=CARTESIAN_POINT ( 'NONE',  ( 17.49862860983166257, -2.500000000000000000, -4.081131818001380474 ) ) ;
#53110=ORIENTED_EDGE ( 'NONE', *, *, #123733, .F. ) ;
#53111=ORIENTED_EDGE ( 'NONE', *, *, #123153, .F. ) ;
#53112=CARTESIAN_POINT ( 'NONE',  ( 10.64999999999990976, 12.50000000000000000, 2.511473670974873507 ) ) ;
#53113=DIRECTION ( 'NONE',  ( -0.000000000000000000, 1.000000000000000000, -0.000000000000000000 ) ) ;
#53114=EDGE_CURVE ( 'NONE', #87285, #46700, #117606, .T. ) ;
#53115=FACE_OUTER_BOUND ( 'NONE', #104694, .T. ) ;
#53116=LINE ( 'NONE', #96093, #74852 ) ;
#53117=FACE_OUTER_BOUND ( 'NONE', #64522, .T. ) ;
#53118=ORIENTED_EDGE ( 'NONE', *, *, #78984, .F. ) ;
#53119=CONICAL_SURFACE ( 'NONE', #28076, 0.1000000000000002554, 0.003490658503988666988 ) ;
#53120=DIRECTION ( 'NONE',  ( -0.000000000000000000, -1.000000000000000000, -0.000000000000000000 ) ) ;
#53121=EDGE_CURVE ( 'NONE', #117879, #75839, #67335, .T. ) ;
#53122=FACE_OUTER_BOUND ( 'NONE', #37251, .T. ) ;
#53123=ORIENTED_EDGE ( 'NONE', *, *, #10108, .T. ) ;
#53124=LINE ( 'NONE', #43314, #51099 ) ;
#53126=EDGE_LOOP ( 'NONE', ( #127364, #76166 ) ) ;
#53127=PLANE ( 'NONE',  #129009 ) ;
#53128=AXIS2_PLACEMENT_3D ( 'NONE', #3659, #73051, #112966 ) ;
#53129=EDGE_LOOP ( 'NONE', ( #37926, #90205 ) ) ;
#53130=CARTESIAN_POINT ( 'NONE',  ( -3.350000000000031619, 12.50000000000000000, -7.188010851410854052 ) ) ;
#53131=DIRECTION ( 'NONE',  ( 0.000000000000000000, -0.9999939076577903929, 0.003490651415223739937 ) ) ;
#53132=ORIENTED_EDGE ( 'NONE', *, *, #72768, .T. ) ;
#53133=ORIENTED_EDGE ( 'NONE', *, *, #101279, .T. ) ;
#53135=DIRECTION ( 'NONE',  ( 0.000000000000000000, 0.000000000000000000, 1.000000000000000000 ) ) ;
#53138=AXIS2_PLACEMENT_3D ( 'NONE', #85779, #45880, #36056 ) ;
#53139=FACE_OUTER_BOUND ( 'NONE', #60771, .T. ) ;
#53140=CIRCLE ( 'NONE', #69866, 0.1000000000000000472 ) ;
#53141=VECTOR ( 'NONE', #79586, 1000.000000000000000 ) ;
#53142=CARTESIAN_POINT ( 'NONE',  ( -9.200000000000006395, 12.50000000000000000, -2.385244779468109755E-15 ) ) ;
#53143=CARTESIAN_POINT ( 'NONE',  ( -1.250000000000001110, 2.500000000000000000, -2.165063509461101710 ) ) ;
#53144=CARTESIAN_POINT ( 'NONE',  ( -11.24999999999996270, 2.500000000000000000, 2.065063509461097624 ) ) ;
#53145=CONICAL_SURFACE ( 'NONE', #59428, 0.09999999999999982514, 0.003490658503988666988 ) ;
#53146=LINE ( 'NONE', #11272, #15000 ) ;
#53147=EDGE_CURVE ( 'NONE', #49253, #32790, #127587, .T. ) ;
#53148=ORIENTED_EDGE ( 'NONE', *, *, #38049, .F. ) ;
#53149=ADVANCED_FACE ( 'NONE', ( #68015 ), #61920, .T. ) ;
#53150=ORIENTED_EDGE ( 'NONE', *, *, #23881, .F. ) ;
#53151=LINE ( 'NONE', #5317, #57026 ) ;
#53152=EDGE_LOOP ( 'NONE', ( #88773, #68707 ) ) ;
#53153=DIRECTION ( 'NONE',  ( 0.000000000000000000, 1.000000000000000000, 0.000000000000000000 ) ) ;
#53154=DIRECTION ( 'NONE',  ( 0.000000000000000000, 1.000000000000000000, 0.000000000000000000 ) ) ;
#53155=CARTESIAN_POINT ( 'NONE',  ( -0.8500000000000386136, 2.500000000000000000, 2.857883832488649301 ) ) ;
#53156=EDGE_LOOP ( 'NONE', ( #79376, #30940, #129311, #118323 ) ) ;
#53157=VERTEX_POINT ( 'NONE', #41001 ) ;
#53158=FACE_BOUND ( 'NONE', #27712, .T. ) ;
#53159=VERTEX_POINT ( 'NONE', #60632 ) ;
#53160=EDGE_CURVE ( 'NONE', #99317, #62165, #100526, .T. ) ;
#53161=CARTESIAN_POINT ( 'NONE',  ( -12.69999999999999396, 2.500000000000000000, -3.983716857408423628 ) ) ;
#53162=DIRECTION ( 'NONE',  ( -0.000000000000000000, 1.000000000000000000, -0.000000000000000000 ) ) ;
#53163=EDGE_CURVE ( 'NONE', #9132, #39516, #52092, .T. ) ;
#53164=CARTESIAN_POINT ( 'NONE',  ( -11.64999999999999680, 2.500000000000000000, 6.395190528383296602 ) ) ;
#53165=DIRECTION ( 'NONE',  ( 0.000000000000000000, -0.000000000000000000, 1.000000000000000000 ) ) ;
#53166=DIRECTION ( 'NONE',  ( 0.000000000000000000, -0.9999939076577903929, 0.003490651415223739937 ) ) ;
#53167=ADVANCED_FACE ( 'NONE', ( #80905 ), #1679, .T. ) ;
#53168=VECTOR ( 'NONE', #37286, 1000.000000000000000 ) ;
#53169=CARTESIAN_POINT ( 'NONE',  ( 2.299999999999948752, 2.500000000000000000, -3.983716857408426293 ) ) ;
#53170=VECTOR ( 'NONE', #45012, 1000.000000000000000 ) ;
#53171=DIRECTION ( 'NONE',  ( -0.000000000000000000, 1.000000000000000000, -0.000000000000000000 ) ) ;
#53172=CARTESIAN_POINT ( 'NONE',  ( 14.14999999999989377, 2.500000000000000000, -2.957883832488653830 ) ) ;
#53173=AXIS2_PLACEMENT_3D ( 'NONE', #114997, #57388, #15511 ) ;
#53174=CIRCLE ( 'NONE', #48970, 0.06509327318403743123 ) ;
#53175=PLANE ( 'NONE',  #91391 ) ;
#53176=DIRECTION ( 'NONE',  ( 0.000000000000000000, 0.000000000000000000, -1.000000000000000000 ) ) ;
#53177=DIRECTION ( 'NONE',  ( 0.000000000000000000, 1.000000000000000000, 0.000000000000000000 ) ) ;
#53178=ADVANCED_FACE ( 'NONE', ( #21323 ), #4750, .T. ) ;
#53179=AXIS2_PLACEMENT_3D ( 'NONE', #15896, #117293, #37499 ) ;
#53180=AXIS2_PLACEMENT_3D ( 'NONE', #105993, #30024, #29380 ) ;
#53181=VERTEX_POINT ( 'NONE', #43574 ) ;
#53182=VERTEX_POINT ( 'NONE', #23251 ) ;
#53183=ORIENTED_EDGE ( 'NONE', *, *, #67077, .F. ) ;
#53184=AXIS2_PLACEMENT_3D ( 'NONE', #111640, #33097, #52708 ) ;
#53185=CARTESIAN_POINT ( 'NONE',  ( -7.900000000000014566, 12.50000000000000000, -3.572213422710612374 ) ) ;
#53186=ORIENTED_EDGE ( 'NONE', *, *, #46162, .T. ) ;
#53187=DIRECTION ( 'NONE',  ( -4.274815082592931898E-19, -0.9999939076577903929, -0.003490651415223739937 ) ) ;
#53188=ORIENTED_EDGE ( 'NONE', *, *, #13914, .F. ) ;
#53189=ORIENTED_EDGE ( 'NONE', *, *, #18097, .T. ) ;
#53190=ORIENTED_EDGE ( 'NONE', *, *, #77498, .F. ) ;
#53191=DIRECTION ( 'NONE',  ( 0.000000000000000000, -0.000000000000000000, 1.000000000000000000 ) ) ;
#53192=VECTOR ( 'NONE', #69956, 1000.000000000000000 ) ;
#53193=AXIS2_PLACEMENT_3D ( 'NONE', #66798, #55065, #94995 ) ;
#53194=CARTESIAN_POINT ( 'NONE',  ( -10.85000000000000142, 12.50000000000000000, 6.560283801567334372 ) ) ;
#53196=CARTESIAN_POINT ( 'NONE',  ( 7.499999999999925393, 2.500000000000000000, -3.537306695894649966 ) ) ;
#53197=LINE ( 'NONE', #42082, #68588 ) ;
#53198=AXIS2_PLACEMENT_3D ( 'NONE', #1848, #41809, #81700 ) ;
#53199=DIRECTION ( 'NONE',  ( 0.000000000000000000, -0.9999939076577903929, 0.003490651415223739937 ) ) ;
#53200=ADVANCED_FACE ( 'NONE', ( #2314 ), #102472, .T. ) ;
#53201=VERTEX_POINT ( 'NONE', #10840 ) ;
#53202=DIRECTION ( 'NONE',  ( 0.000000000000000000, 1.000000000000000000, 0.000000000000000000 ) ) ;
#53203=EDGE_LOOP ( 'NONE', ( #52549, #60675 ) ) ;
#53204=ORIENTED_EDGE ( 'NONE', *, *, #85323, .T. ) ;
#53205=VERTEX_POINT ( 'NONE', #101186 ) ;
#53206=PLANE ( 'NONE',  #421 ) ;
#53207=ORIENTED_EDGE ( 'NONE', *, *, #118599, .F. ) ;
#53208=ORIENTED_EDGE ( 'NONE', *, *, #36444, .F. ) ;
#53209=VERTEX_POINT ( 'NONE', #41649 ) ;
#53210=CIRCLE ( 'NONE', #28154, 0.06509327318403745899 ) ;
#53211=FACE_OUTER_BOUND ( 'NONE', #102114, .T. ) ;
#53212=PLANE ( 'NONE',  #120760 ) ;
#53213=CARTESIAN_POINT ( 'NONE',  ( 5.799999999999934985, 12.50000000000000000, -4.330127018922201643 ) ) ;
#53214=EDGE_CURVE ( 'NONE', #11848, #69557, #22001, .T. ) ;
#53215=CARTESIAN_POINT ( 'NONE',  ( 13.34999999999989662, 12.50000000000000000, -1.472243186433550122 ) ) ;
#53216=DIRECTION ( 'NONE',  ( -0.000000000000000000, -1.000000000000000000, -0.000000000000000000 ) ) ;
#53218=PLANE ( 'NONE',  #67720 ) ;
#53219=AXIS2_PLACEMENT_3D ( 'NONE', #103209, #33202, #73110 ) ;
#53220=AXIS2_PLACEMENT_3D ( 'NONE', #38651, #68720, #108002 ) ;
#53221=VERTEX_POINT ( 'NONE', #71077 ) ;
#53222=FACE_OUTER_BOUND ( 'NONE', #84917, .T. ) ;
#53223=ORIENTED_EDGE ( 'NONE', *, *, #63674, .F. ) ;
#53225=EDGE_LOOP ( 'NONE', ( #67640, #74397 ) ) ;
#53226=EDGE_CURVE ( 'NONE', #68394, #68963, #107163, .T. ) ;
#53227=VERTEX_POINT ( 'NONE', #33729 ) ;
#53228=DIRECTION ( 'NONE',  ( -0.000000000000000000, -1.000000000000000000, -0.000000000000000000 ) ) ;
#53229=DIRECTION ( 'NONE',  ( 0.000000000000000000, 0.000000000000000000, 1.000000000000000000 ) ) ;
#53230=CIRCLE ( 'NONE', #61543, 0.1000000000000002554 ) ;
#53231=LINE ( 'NONE', #13277, #36282 ) ;
#53232=AXIS2_PLACEMENT_3D ( 'NONE', #86446, #104785, #14470 ) ;
#53233=EDGE_LOOP ( 'NONE', ( #102225, #57110, #96233, #74007 ) ) ;
#53234=EDGE_LOOP ( 'NONE', ( #86958, #2419 ) ) ;
#53235=CARTESIAN_POINT ( 'NONE',  ( 7.499999999999960032, 2.500000000000000000, 0.09999999999999772959 ) ) ;
#53236=DIRECTION ( 'NONE',  ( -4.274815082592931898E-19, -0.9999939076577903929, -0.003490651415223739937 ) ) ;
#53237=CARTESIAN_POINT ( 'NONE',  ( 6.849999999999930367, 12.50000000000000000, -6.841600689897078702 ) ) ;
#53238=LINE ( 'NONE', #70934, #107810 ) ;
#53239=DIRECTION ( 'NONE',  ( 0.000000000000000000, 0.000000000000000000, 1.000000000000000000 ) ) ;
#53240=ORIENTED_EDGE ( 'NONE', *, *, #52525, .T. ) ;
#53241=CONICAL_SURFACE ( 'NONE', #128568, 0.1000000000000002554, 0.003490658503988666988 ) ;
#53242=AXIS2_PLACEMENT_3D ( 'NONE', #57331, #79552, #97248 ) ;
#53243=CARTESIAN_POINT ( 'NONE',  ( 8.149999999999920419, 2.500000000000000000, -2.511473670974877948 ) ) ;
#53244=VECTOR ( 'NONE', #33521, 1000.000000000000000 ) ;
#53245=ORIENTED_EDGE ( 'NONE', *, *, #34044, .T. ) ;
#53246=AXIS2_PLACEMENT_3D ( 'NONE', #65822, #34458, #16065 ) ;
#53247=DIRECTION ( 'NONE',  ( 0.000000000000000000, 1.000000000000000000, 0.000000000000000000 ) ) ;
#53248=EDGE_CURVE ( 'NONE', #24257, #77451, #12142, .T. ) ;
#53250=CARTESIAN_POINT ( 'NONE',  ( 2.899999999999946620, 2.500000000000000000, 0.7928203230275495672 ) ) ;
#53251=CARTESIAN_POINT ( 'NONE',  ( 2.299999999999948752, 2.500000000000000000, -3.983716857408426293 ) ) ;
#53252=CARTESIAN_POINT ( 'NONE',  ( 2.499999999999947153, 2.500000000000000000, -3.537306695894649966 ) ) ;
#53253=DIRECTION ( 'NONE',  ( -4.274815082592931898E-19, -0.9999939076577903929, -0.003490651415223739937 ) ) ;
#53254=ORIENTED_EDGE ( 'NONE', *, *, #88836, .F. ) ;
#53255=ADVANCED_FACE ( 'NONE', ( #112300 ), #123988, .T. ) ;
#53256=CARTESIAN_POINT ( 'NONE',  ( -7.300000000000013145, 12.50000000000000000, 3.983716857408420076 ) ) ;
#53257=VECTOR ( 'NONE', #110522, 1000.000000000000000 ) ;
#53258=CARTESIAN_POINT ( 'NONE',  ( -4.150000000000027889, 2.500000000000000000, -6.495190528383302464 ) ) ;
#53259=DIRECTION ( 'NONE',  ( 0.000000000000000000, 0.000000000000000000, 1.000000000000000000 ) ) ;
#53260=CONICAL_SURFACE ( 'NONE', #90900, 0.1000000000000000472, 0.003490658503988666988 ) ;
#53262=AXIS2_PLACEMENT_3D ( 'NONE', #35662, #54014, #65096 ) ;
#53263=EDGE_CURVE ( 'NONE', #76531, #92529, #75865, .T. ) ;
#53264=ADVANCED_FACE ( 'NONE', ( #61268 ), #62564, .T. ) ;
#53265=EDGE_CURVE ( 'NONE', #112003, #67433, #103064, .T. ) ;
#53266=ADVANCED_FACE ( 'NONE', ( #12781 ), #73816, .T. ) ;
#53267=DIRECTION ( 'NONE',  ( -0.000000000000000000, 1.000000000000000000, -0.000000000000000000 ) ) ;
#53269=AXIS2_PLACEMENT_3D ( 'NONE', #72650, #102722, #41264 ) ;
#53270=ORIENTED_EDGE ( 'NONE', *, *, #87681, .T. ) ;
#53271=VECTOR ( 'NONE', #89262, 1000.000000000000000 ) ;
#53272=EDGE_CURVE ( 'NONE', #76489, #95522, #119785, .T. ) ;
#53273=CARTESIAN_POINT ( 'NONE',  ( -1.050000000000038236, 12.50000000000000000, -6.148780366869526226 ) ) ;
#53274=ADVANCED_FACE ( 'NONE', ( #55311 ), #75577, .T. ) ;
#53275=CIRCLE ( 'NONE', #63731, 0.1000000000000002554 ) ;
#53276=VERTEX_POINT ( 'NONE', #104406 ) ;
#53277=CARTESIAN_POINT ( 'NONE',  ( 15.86953761859728118, -2.463355995079595129, -3.896699429482295418 ) ) ;
#53278=CARTESIAN_POINT ( 'NONE',  ( 8.749999999999921840, 2.500000000000000000, -5.802370205355749988 ) ) ;
#53279=EDGE_CURVE ( 'NONE', #12586, #3575, #2698, .T. ) ;
#53280=DIRECTION ( 'NONE',  ( -0.000000000000000000, -1.000000000000000000, -0.000000000000000000 ) ) ;
#53281=ORIENTED_EDGE ( 'NONE', *, *, #63713, .T. ) ;
#53282=EDGE_CURVE ( 'NONE', #13086, #35232, #109320, .T. ) ;
#53283=AXIS2_PLACEMENT_3D ( 'NONE', #45010, #103922, #14233 ) ;
#53284=AXIS2_PLACEMENT_3D ( 'NONE', #102082, #22888, #12398 ) ;
#53285=DIRECTION ( 'NONE',  ( 0.000000000000000000, 1.000000000000000000, 0.000000000000000000 ) ) ;
#53286=EDGE_CURVE ( 'NONE', #18475, #11947, #46128, .T. ) ;
#53287=DIRECTION ( 'NONE',  ( 0.000000000000000000, 1.000000000000000000, 0.000000000000000000 ) ) ;
#53288=CIRCLE ( 'NONE', #109718, 0.06509327318403745899 ) ;
#53289=EDGE_CURVE ( 'NONE', #57293, #13968, #4851, .T. ) ;
#53290=EDGE_LOOP ( 'NONE', ( #121243, #45815, #49721, #125511 ) ) ;
#53291=ORIENTED_EDGE ( 'NONE', *, *, #85722, .F. ) ;
#53292=ORIENTED_EDGE ( 'NONE', *, *, #56026, .T. ) ;
#53293=CARTESIAN_POINT ( 'NONE',  ( -5.400000000000019895, 2.500000000000000000, 3.537306695894645081 ) ) ;
#53294=DIRECTION ( 'NONE',  ( -0.000000000000000000, 1.000000000000000000, -0.000000000000000000 ) ) ;
#53295=LINE ( 'NONE', #40912, #67212 ) ;
#53296=ORIENTED_EDGE ( 'NONE', *, *, #55506, .F. ) ;
#53297=DIRECTION ( 'NONE',  ( 0.000000000000000000, 0.000000000000000000, -1.000000000000000000 ) ) ;
#53298=CARTESIAN_POINT ( 'NONE',  ( -5.200000000000022382, 2.500000000000000000, 4.676537180435972552 ) ) ;
#53299=CIRCLE ( 'NONE', #97195, 0.06509327318403745899 ) ;
#53300=VERTEX_POINT ( 'NONE', #54021 ) ;
#53301=FACE_OUTER_BOUND ( 'NONE', #114451, .T. ) ;
#53302=DIRECTION ( 'NONE',  ( 0.000000000000000000, -0.9999939076577903929, 0.003490651415223739937 ) ) ;
#53303=DIRECTION ( 'NONE',  ( -0.000000000000000000, -1.000000000000000000, -0.000000000000000000 ) ) ;
#53304=CARTESIAN_POINT ( 'NONE',  ( 2.699999999999947331, 2.500000000000000000, -0.4464101615137783252 ) ) ;
#53305=DIRECTION ( 'NONE',  ( -0.000000000000000000, 1.000000000000000000, -0.000000000000000000 ) ) ;
#53306=LINE ( 'NONE', #12071, #59765 ) ;
#53307=DIRECTION ( 'NONE',  ( 0.000000000000000000, -0.000000000000000000, 1.000000000000000000 ) ) ;
#53308=AXIS2_PLACEMENT_3D ( 'NONE', #93248, #31118, #102420 ) ;
#53309=AXIS2_PLACEMENT_3D ( 'NONE', #109795, #127503, #110427 ) ;
#53310=ORIENTED_EDGE ( 'NONE', *, *, #50975, .F. ) ;
#53311=ORIENTED_EDGE ( 'NONE', *, *, #9492, .T. ) ;
#53312=ORIENTED_EDGE ( 'NONE', *, *, #123634, .T. ) ;
#53313=ORIENTED_EDGE ( 'NONE', *, *, #64158, .T. ) ;
#53314=DIRECTION ( 'NONE',  ( -4.274815082592931898E-19, -0.9999939076577903929, -0.003490651415223739937 ) ) ;
#53315=CARTESIAN_POINT ( 'NONE',  ( -11.84999999999999787, 2.500000000000000000, -6.841600689897074261 ) ) ;
#53316=DIRECTION ( 'NONE',  ( 0.000000000000000000, -0.9999939076577903929, 0.003490651415223739937 ) ) ;
#53317=ORIENTED_EDGE ( 'NONE', *, *, #107023, .T. ) ;
#53318=FACE_BOUND ( 'NONE', #94798, .T. ) ;
#53319=FACE_OUTER_BOUND ( 'NONE', #106323, .T. ) ;
#53320=DIRECTION ( 'NONE',  ( 0.000000000000000000, 0.000000000000000000, -1.000000000000000000 ) ) ;
#53321=AXIS2_PLACEMENT_3D ( 'NONE', #102364, #63072, #45382 ) ;
#53322=EDGE_CURVE ( 'NONE', #79354, #64399, #80088, .T. ) ;
#53323=CARTESIAN_POINT ( 'NONE',  ( 5.649999999999934630, 2.500000000000000000, -2.511473670974877948 ) ) ;
#53324=DIRECTION ( 'NONE',  ( -0.000000000000000000, 1.000000000000000000, -0.000000000000000000 ) ) ;
#53325=CIRCLE ( 'NONE', #26125, 0.1000000000000000056 ) ;
#53326=EDGE_CURVE ( 'NONE', #124333, #103811, #50840, .T. ) ;
#53327=CARTESIAN_POINT ( 'NONE',  ( 13.94999999999989626, 2.500000000000000000, 2.611473670974873151 ) ) ;
#53328=FACE_OUTER_BOUND ( 'NONE', #33357, .T. ) ;
#53329=DIRECTION ( 'NONE',  ( -4.274815082592931898E-19, -0.9999939076577903929, -0.003490651415223739937 ) ) ;
#53330=DIRECTION ( 'NONE',  ( -0.000000000000000000, -1.000000000000000000, -0.000000000000000000 ) ) ;
#53331=CARTESIAN_POINT ( 'NONE',  ( -5.200000000000024158, 12.50000000000000000, -4.611443907251939756 ) ) ;
#53332=ADVANCED_FACE ( 'NONE', ( #86697 ), #6187, .T. ) ;
#53333=ORIENTED_EDGE ( 'NONE', *, *, #8213, .F. ) ;
#53334=AXIS2_PLACEMENT_3D ( 'NONE', #42857, #4164, #121373 ) ;
#53335=EDGE_LOOP ( 'NONE', ( #118263, #71263 ) ) ;
#53336=ORIENTED_EDGE ( 'NONE', *, *, #51625, .F. ) ;
#53337=EDGE_LOOP ( 'NONE', ( #35210, #69455 ) ) ;
#53338=ORIENTED_EDGE ( 'NONE', *, *, #103488, .T. ) ;
#53339=ORIENTED_EDGE ( 'NONE', *, *, #73652, .T. ) ;
#53340=DIRECTION ( 'NONE',  ( -0.000000000000000000, -1.000000000000000000, -0.000000000000000000 ) ) ;
#53341=ORIENTED_EDGE ( 'NONE', *, *, #45619, .T. ) ;
#53342=VERTEX_POINT ( 'NONE', #14067 ) ;
#53343=DIRECTION ( 'NONE',  ( -0.000000000000000000, 1.000000000000000000, -0.000000000000000000 ) ) ;
#53344=DIRECTION ( 'NONE',  ( 0.000000000000000000, 1.000000000000000000, 0.000000000000000000 ) ) ;
#53345=CARTESIAN_POINT ( 'NONE',  ( -4.150000000000025224, 2.500000000000000000, 6.395190528383296602 ) ) ;
#53346=CIRCLE ( 'NONE', #86773, 0.1000000000000002554 ) ;
#53347=ORIENTED_EDGE ( 'NONE', *, *, #123702, .T. ) ;
#53348=DIRECTION ( 'NONE',  ( 0.000000000000000000, 1.000000000000000000, 0.000000000000000000 ) ) ;
#53349=ORIENTED_EDGE ( 'NONE', *, *, #94325, .F. ) ;
#53350=AXIS2_PLACEMENT_3D ( 'NONE', #109659, #101123, #31745 ) ;
#53351=ORIENTED_EDGE ( 'NONE', *, *, #34956, .T. ) ;
#53352=DIRECTION ( 'NONE',  ( 0.000000000000000000, -0.000000000000000000, 1.000000000000000000 ) ) ;
#53353=AXIS2_PLACEMENT_3D ( 'NONE', #47222, #46554, #96299 ) ;
#53354=CARTESIAN_POINT ( 'NONE',  ( -10.40000000000000213, 2.500000000000000000, -4.330127018922197202 ) ) ;
#53355=ORIENTED_EDGE ( 'NONE', *, *, #69459, .F. ) ;
#53356=EDGE_LOOP ( 'NONE', ( #27540, #23682 ) ) ;
#53357=CARTESIAN_POINT ( 'NONE',  ( -9.350000000000004974, 12.50000000000000000, 6.906693963081109722 ) ) ;
#53359=VECTOR ( 'NONE', #86522, 1000.000000000000000 ) ;
#53360=CARTESIAN_POINT ( 'NONE',  ( 8.549999999999918998, 2.500000000000000000, 6.941600689897073018 ) ) ;
#53362=CARTESIAN_POINT ( 'NONE',  ( 4.999999999999936939, 2.500000000000000000, -3.637306695894650055 ) ) ;
#53363=AXIS2_PLACEMENT_3D ( 'NONE', #49549, #89459, #129418 ) ;
#53364=DIRECTION ( 'NONE',  ( 0.000000000000000000, 1.000000000000000000, 0.000000000000000000 ) ) ;
#53365=EDGE_CURVE ( 'NONE', #36522, #129616, #92607, .T. ) ;
#53366=ORIENTED_EDGE ( 'NONE', *, *, #41575, .F. ) ;
#53367=CARTESIAN_POINT ( 'NONE',  ( 15.62876697814516369, -2.500000000000000000, 5.624417669420343380 ) ) ;
#53368=AXIS2_PLACEMENT_3D ( 'NONE', #41654, #30539, #70442 ) ;
#53370=EDGE_LOOP ( 'NONE', ( #104674, #127454 ) ) ;
#53371=FACE_OUTER_BOUND ( 'NONE', #89401, .T. ) ;
#53372=ORIENTED_EDGE ( 'NONE', *, *, #14086, .F. ) ;
#53373=DIRECTION ( 'NONE',  ( 0.000000000000000000, 0.000000000000000000, 1.000000000000000000 ) ) ;
#53374=DIRECTION ( 'NONE',  ( 0.000000000000000000, 1.000000000000000000, 0.000000000000000000 ) ) ;
#53375=CIRCLE ( 'NONE', #74202, 0.06509327318403745899 ) ;
#53376=EDGE_CURVE ( 'NONE', #121167, #94312, #6889, .T. ) ;
#53377=CARTESIAN_POINT ( 'NONE',  ( 0.3999999999999563904, 2.500000000000000000, 3.737306695894644371 ) ) ;
#53378=EDGE_CURVE ( 'NONE', #64213, #79919, #78024, .T. ) ;
#53379=CARTESIAN_POINT ( 'NONE',  ( -0.6500000000000398792, 2.500000000000000000, -6.941600689897078347 ) ) ;
#53380=EDGE_LOOP ( 'NONE', ( #21047, #52416 ) ) ;
#53381=CARTESIAN_POINT ( 'NONE',  ( -7.500000000000013323, 12.50000000000000000, 5.088040615133786027 ) ) ;
#53382=DIRECTION ( 'NONE',  ( 0.000000000000000000, 0.000000000000000000, -1.000000000000000000 ) ) ;
#53383=EDGE_LOOP ( 'NONE', ( #116609, #116170, #59249, #31453 ) ) ;
#53384=EDGE_LOOP ( 'NONE', ( #67782, #125109 ) ) ;
#53385=EDGE_CURVE ( 'NONE', #43544, #106720, #8961, .T. ) ;
#53386=ORIENTED_EDGE ( 'NONE', *, *, #35732, .T. ) ;
#53387=CARTESIAN_POINT ( 'NONE',  ( 5.849999999999935696, 2.500000000000000000, -6.495190528383302464 ) ) ;
#53389=AXIS2_PLACEMENT_3D ( 'NONE', #112071, #52492, #92418 ) ;
#53390=DIRECTION ( 'NONE',  ( 0.000000000000000000, -0.9999939076577903929, 0.003490651415223739937 ) ) ;
#53391=DIRECTION ( 'NONE',  ( -0.000000000000000000, 1.000000000000000000, -0.000000000000000000 ) ) ;
#53392=CARTESIAN_POINT ( 'NONE',  ( 8.349999999999919709, 2.500000000000000000, 6.495190528383297135 ) ) ;
#53393=DIRECTION ( 'NONE',  ( 0.000000000000000000, 0.000000000000000000, -1.000000000000000000 ) ) ;
#53394=AXIS2_PLACEMENT_3D ( 'NONE', #110138, #32248, #40782 ) ;
#53395=AXIS2_PLACEMENT_3D ( 'NONE', #24475, #61838, #72300 ) ;
#53396=EDGE_LOOP ( 'NONE', ( #54612, #44983 ) ) ;
#53397=AXIS2_PLACEMENT_3D ( 'NONE', #15431, #46858, #14771 ) ;
#53398=FACE_OUTER_BOUND ( 'NONE', #66171, .T. ) ;
#53399=EDGE_CURVE ( 'NONE', #119766, #88678, #44576, .T. ) ;
#53400=ORIENTED_EDGE ( 'NONE', *, *, #93369, .F. ) ;
#53401=CARTESIAN_POINT ( 'NONE',  ( 5.849999999999933920, 2.500000000000000000, 6.595190528383296780 ) ) ;
#53402=DIRECTION ( 'NONE',  ( 0.000000000000000000, -0.000000000000000000, 1.000000000000000000 ) ) ;
#53403=LINE ( 'NONE', #14730, #79833 ) ;
#53404=DIRECTION ( 'NONE',  ( 0.000000000000000000, -0.000000000000000000, 1.000000000000000000 ) ) ;
#53405=ORIENTED_EDGE ( 'NONE', *, *, #10823, .F. ) ;
#53406=CIRCLE ( 'NONE', #26209, 0.1000000000000000472 ) ;
#53407=EDGE_CURVE ( 'NONE', #101832, #92344, #67537, .T. ) ;
#53408=AXIS2_PLACEMENT_3D ( 'NONE', #128843, #118339, #28682 ) ;
#53409=CARTESIAN_POINT ( 'NONE',  ( -9.600000000000006750, 12.50000000000000000, 0.7579135962115869374 ) ) ;
#53410=LINE ( 'NONE', #100560, #58849 ) ;
#53411=VERTEX_POINT ( 'NONE', #76883 ) ;
#53412=EDGE_CURVE ( 'NONE', #104601, #32860, #125337, .T. ) ;
#53413=ADVANCED_FACE ( 'NONE', ( #24555 ), #117708, .T. ) ;
#53414=EDGE_CURVE ( 'NONE', #12173, #87251, #38328, .T. ) ;
#53415=EDGE_CURVE ( 'NONE', #19409, #15503, #13154, .T. ) ;
#53416=EDGE_LOOP ( 'NONE', ( #58798, #46727 ) ) ;
#53417=DIRECTION ( 'NONE',  ( 0.000000000000000000, 0.000000000000000000, 1.000000000000000000 ) ) ;
#53418=AXIS2_PLACEMENT_3D ( 'NONE', #125250, #15921, #65672 ) ;
#53419=AXIS2_PLACEMENT_3D ( 'NONE', #16584, #4186, #114797 ) ;
#53420=ORIENTED_EDGE ( 'NONE', *, *, #52214, .T. ) ;
#53422=CARTESIAN_POINT ( 'NONE',  ( 10.39999999999990976, 2.500000000000000000, 4.430127018922196847 ) ) ;
#53423=EDGE_CURVE ( 'NONE', #112989, #73598, #107265, .T. ) ;
#53424=EDGE_CURVE ( 'NONE', #16575, #87037, #647, .T. ) ;
#53425=VERTEX_POINT ( 'NONE', #9432 ) ;
#53426=CARTESIAN_POINT ( 'NONE',  ( 17.88933034088960028, 0.4802206367767866690, -4.999988745079795294 ) ) ;
#53427=CARTESIAN_POINT ( 'NONE',  ( -5.000000000000024869, 2.500000000000000000, -4.922947341949753586 ) ) ;
#53428=DIRECTION ( 'NONE',  ( -0.000000000000000000, -1.000000000000000000, -0.000000000000000000 ) ) ;
#53429=EDGE_LOOP ( 'NONE', ( #38755, #24337, #123514, #24574 ) ) ;
#53430=EDGE_CURVE ( 'NONE', #58340, #52125, #15309, .T. ) ;
#53431=AXIS2_PLACEMENT_3D ( 'NONE', #120307, #79732, #30648 ) ;
#53432=DIRECTION ( 'NONE',  ( -0.000000000000000000, -1.000000000000000000, -0.000000000000000000 ) ) ;
#53434=ORIENTED_EDGE ( 'NONE', *, *, #32619, .F. ) ;
#53435=CARTESIAN_POINT ( 'NONE',  ( 17.45053073489854967, 1.969617801099436738, 4.507369966539876316 ) ) ;
#53436=EDGE_CURVE ( 'NONE', #42825, #120364, #10075, .T. ) ;
#53437=DIRECTION ( 'NONE',  ( -0.000000000000000000, 1.000000000000000000, -0.000000000000000000 ) ) ;
#53438=CIRCLE ( 'NONE', #70160, 0.1000000000000002554 ) ;
#53439=EDGE_CURVE ( 'NONE', #17385, #47052, #61309, .T. ) ;
#53440=ORIENTED_EDGE ( 'NONE', *, *, #97279, .F. ) ;
#53441=CIRCLE ( 'NONE', #74355, 0.09999999999999982514 ) ;
#53442=EDGE_LOOP ( 'NONE', ( #99366, #32130, #17332, #117815 ) ) ;
#53443=VECTOR ( 'NONE', #95736, 1000.000000000000000 ) ;
#53444=ORIENTED_EDGE ( 'NONE', *, *, #119902, .T. ) ;
#53445=VERTEX_POINT ( 'NONE', #238 ) ;
#53446=FACE_OUTER_BOUND ( 'NONE', #126495, .T. ) ;
#53447=CARTESIAN_POINT ( 'NONE',  ( 12.09999999999990195, 2.500000000000000000, 0.6928203230275494784 ) ) ;
#53448=DIRECTION ( 'NONE',  ( -0.000000000000000000, 1.000000000000000000, -0.000000000000000000 ) ) ;
#53449=FACE_BOUND ( 'NONE', #27628, .T. ) ;
#53450=EDGE_LOOP ( 'NONE', ( #3697, #96545, #54493, #115342 ) ) ;
#53452=CARTESIAN_POINT ( 'NONE',  ( -6.650000000000018119, 2.500000000000000000, -2.165063509461101710 ) ) ;
#53453=DIRECTION ( 'NONE',  ( 0.000000000000000000, 1.000000000000000000, 0.000000000000000000 ) ) ;
#53454=CIRCLE ( 'NONE', #88951, 0.06509327318403745899 ) ;
#53455=CARTESIAN_POINT ( 'NONE',  ( 1.899999999999951283, 12.50000000000000000, -4.741630453620015118 ) ) ;
#53456=DIRECTION ( 'NONE',  ( 0.000000000000000000, 0.000000000000000000, 1.000000000000000000 ) ) ;
#53457=LINE ( 'NONE', #93373, #65901 ) ;
#53458=VECTOR ( 'NONE', #11363, 1000.000000000000000 ) ;
#53459=AXIS2_PLACEMENT_3D ( 'NONE', #97099, #87264, #37547 ) ;
#53460=DIRECTION ( 'NONE',  ( 0.000000000000000000, 0.000000000000000000, 1.000000000000000000 ) ) ;
#53462=ORIENTED_EDGE ( 'NONE', *, *, #61669, .T. ) ;
#53463=EDGE_LOOP ( 'NONE', ( #43492, #95357, #110868, #100899 ) ) ;
#53464=ORIENTED_EDGE ( 'NONE', *, *, #117787, .F. ) ;
#53465=EDGE_LOOP ( 'NONE', ( #71405, #67303 ) ) ;
#53466=AXIS2_PLACEMENT_3D ( 'NONE', #113268, #34078, #94268 ) ;
#53467=VERTEX_POINT ( 'NONE', #48076 ) ;
#53468=DIRECTION ( 'NONE',  ( 0.000000000000000000, 1.000000000000000000, 0.000000000000000000 ) ) ;
#53469=DIRECTION ( 'NONE',  ( 0.000000000000000000, 0.000000000000000000, 1.000000000000000000 ) ) ;
#53470=VERTEX_POINT ( 'NONE', #118733 ) ;
#53471=FACE_BOUND ( 'NONE', #107439, .T. ) ;
#53472=DIRECTION ( 'NONE',  ( -0.000000000000000000, -1.000000000000000000, -0.000000000000000000 ) ) ;
#53473=EDGE_CURVE ( 'NONE', #9353, #127509, #67691, .T. ) ;
#53474=ADVANCED_FACE ( 'NONE', ( #97802 ), #57089, .T. ) ;
#53475=ORIENTED_EDGE ( 'NONE', *, *, #85880, .T. ) ;
#53476=LINE ( 'NONE', #25269, #124764 ) ;
#53477=DIRECTION ( 'NONE',  ( 0.000000000000000000, 0.000000000000000000, -1.000000000000000000 ) ) ;
#53478=DIRECTION ( 'NONE',  ( 0.000000000000000000, -0.9999939076577903929, 0.003490651415223739937 ) ) ;
#53479=VECTOR ( 'NONE', #71325, 1000.000000000000000 ) ;
#53480=ORIENTED_EDGE ( 'NONE', *, *, #127488, .F. ) ;
#53481=FACE_OUTER_BOUND ( 'NONE', #48879, .T. ) ;
#53482=ORIENTED_EDGE ( 'NONE', *, *, #103551, .T. ) ;
#53483=EDGE_LOOP ( 'NONE', ( #5529, #82362, #65578, #124827 ) ) ;
#53484=ORIENTED_EDGE ( 'NONE', *, *, #60044, .F. ) ;
#53485=DIRECTION ( 'NONE',  ( 0.000000000000000000, 0.000000000000000000, 1.000000000000000000 ) ) ;
#53486=DIRECTION ( 'NONE',  ( 0.000000000000000000, 1.000000000000000000, 0.000000000000000000 ) ) ;
#53487=CIRCLE ( 'NONE', #34724, 0.06509327318403741736 ) ;
#53488=CARTESIAN_POINT ( 'NONE',  ( -15.59999999999998010, 2.500000000000000000, 0.3464101615137759604 ) ) ;
#53489=ORIENTED_EDGE ( 'NONE', *, *, #5778, .F. ) ;
#53490=DIRECTION ( 'NONE',  ( -4.274815082592931898E-19, -0.9999939076577903929, -0.003490651415223739937 ) ) ;
#53491=AXIS2_PLACEMENT_3D ( 'NONE', #105620, #76159, #25113 ) ;
#53492=LINE ( 'NONE', #15475, #76246 ) ;
#53493=VECTOR ( 'NONE', #42220, 1000.000000000000000 ) ;
#53494=DIRECTION ( 'NONE',  ( -0.000000000000000000, -1.000000000000000000, -0.000000000000000000 ) ) ;
#53496=ORIENTED_EDGE ( 'NONE', *, *, #32013, .T. ) ;
#53497=LINE ( 'NONE', #122879, #101818 ) ;
#53498=VERTEX_POINT ( 'NONE', #67032 ) ;
#53499=CARTESIAN_POINT ( 'NONE',  ( -6.450000000000016165, 2.500000000000000000, 6.741600689897071952 ) ) ;
#53500=VECTOR ( 'NONE', #49744, 1000.000000000000000 ) ;
#53501=ORIENTED_EDGE ( 'NONE', *, *, #16341, .T. ) ;
#53502=CONICAL_SURFACE ( 'NONE', #13767, 0.1000000000000000472, 0.003490658503988666988 ) ;
#53503=AXIS2_PLACEMENT_3D ( 'NONE', #110776, #7577, #88049 ) ;
#53504=ORIENTED_EDGE ( 'NONE', *, *, #59365, .F. ) ;
#53506=CARTESIAN_POINT ( 'NONE',  ( -10.20000000000000462, 2.500000000000000000, -4.676537180435973440 ) ) ;
#53507=DIRECTION ( 'NONE',  ( -0.000000000000000000, -1.000000000000000000, -0.000000000000000000 ) ) ;
#53508=DIRECTION ( 'NONE',  ( 0.000000000000000000, -0.000000000000000000, 1.000000000000000000 ) ) ;
#53509=CARTESIAN_POINT ( 'NONE',  ( 9.399999999999915090, 2.500000000000000000, -4.083716857408426826 ) ) ;
#53510=VERTEX_POINT ( 'NONE', #8127 ) ;
#53511=ORIENTED_EDGE ( 'NONE', *, *, #55964, .T. ) ;
#53512=EDGE_CURVE ( 'NONE', #64031, #91293, #86324, .T. ) ;
#53513=DIRECTION ( 'NONE',  ( -0.000000000000000000, -1.000000000000000000, -0.000000000000000000 ) ) ;
#53515=AXIS2_PLACEMENT_3D ( 'NONE', #51248, #22431, #91150 ) ;
#53516=FACE_OUTER_BOUND ( 'NONE', #76318, .T. ) ;
#53517=DIRECTION ( 'NONE',  ( 0.000000000000000000, 0.000000000000000000, 1.000000000000000000 ) ) ;
#53518=VERTEX_POINT ( 'NONE', #47430 ) ;
#53519=ORIENTED_EDGE ( 'NONE', *, *, #52955, .T. ) ;
#53520=DIRECTION ( 'NONE',  ( 0.000000000000000000, 1.000000000000000000, 0.000000000000000000 ) ) ;
#53521=ORIENTED_EDGE ( 'NONE', *, *, #104362, .T. ) ;
#53522=EDGE_CURVE ( 'NONE', #48111, #4340, #15211, .T. ) ;
#53523=CARTESIAN_POINT ( 'NONE',  ( -4.800000000000026468, 2.500000000000000000, -4.676537180435978769 ) ) ;
#53524=DIRECTION ( 'NONE',  ( 0.000000000000000000, 1.000000000000000000, 0.000000000000000000 ) ) ;
#53525=ORIENTED_EDGE ( 'NONE', *, *, #28119, .T. ) ;
#53526=CARTESIAN_POINT ( 'NONE',  ( -6.050000000000022027, 2.500000000000000000, -1.818653347947326138 ) ) ;
#53527=CARTESIAN_POINT ( 'NONE',  ( -11.24999999999999822, 2.500000000000000000, 1.372243186433545370 ) ) ;
#53528=CARTESIAN_POINT ( 'NONE',  ( -9.150000000000009237, 2.500000000000000000, 1.372243186433545370 ) ) ;
#53529=CARTESIAN_POINT ( 'NONE',  ( -7.100000000000018296, 2.500000000000000000, -4.330127018922201643 ) ) ;
#53530=EDGE_CURVE ( 'NONE', #124307, #129616, #87326, .T. ) ;
#53531=EDGE_CURVE ( 'NONE', #58192, #105776, #48791, .T. ) ;
#53532=CARTESIAN_POINT ( 'NONE',  ( -13.34999999999999076, 2.500000000000000000, 2.265063509461101354 ) ) ;
#53533=ORIENTED_EDGE ( 'NONE', *, *, #77370, .F. ) ;
#53534=DIRECTION ( 'NONE',  ( 0.000000000000000000, 0.000000000000000000, -1.000000000000000000 ) ) ;
#53535=VECTOR ( 'NONE', #106036, 1000.000000000000000 ) ;
#53536=CARTESIAN_POINT ( 'NONE',  ( 76.45227062015452191, -3.905198618276467304, 5.870121734768856570 ) ) ;
#53537=ORIENTED_EDGE ( 'NONE', *, *, #61888, .F. ) ;
#53538=ORIENTED_EDGE ( 'NONE', *, *, #41781, .T. ) ;
#53539=EDGE_CURVE ( 'NONE', #180, #45027, #105213, .T. ) ;
#53542=DIRECTION ( 'NONE',  ( -0.000000000000000000, -1.000000000000000000, -0.000000000000000000 ) ) ;
#53543=CARTESIAN_POINT ( 'NONE',  ( -2.900000000000029221, 2.500000000000000000, -4.430127018922202176 ) ) ;
#53544=CARTESIAN_POINT ( 'NONE',  ( -3.950000000000026379, 12.50000000000000000, -1.818653347947326138 ) ) ;
#53545=CARTESIAN_POINT ( 'NONE',  ( -9.400000000000007461, 2.500000000000000000, 4.576537180435972019 ) ) ;
#53546=LINE ( 'NONE', #4400, #128303 ) ;
#53547=CARTESIAN_POINT ( 'NONE',  ( -7.950000000000009059, 2.500000000000000000, 6.495190528383297135 ) ) ;
#53548=LINE ( 'NONE', #93466, #72891 ) ;
#53549=CARTESIAN_POINT ( 'NONE',  ( -12.49999999999995914, 2.500000000000000000, -0.09999999999999815981 ) ) ;
#53550=CARTESIAN_POINT ( 'NONE',  ( 1.649999999999951950, 12.50000000000000000, -5.867463478539787225 ) ) ;
#53551=CONICAL_SURFACE ( 'NONE', #78694, 0.1000000000000002554, 0.003490658503988666988 ) ;
#53552=EDGE_LOOP ( 'NONE', ( #94915, #112954 ) ) ;
#53553=VERTEX_POINT ( 'NONE', #77517 ) ;
#53554=ORIENTED_EDGE ( 'NONE', *, *, #97906, .T. ) ;
#53555=ORIENTED_EDGE ( 'NONE', *, *, #58245, .T. ) ;
#53556=DIRECTION ( 'NONE',  ( 0.000000000000000000, 0.000000000000000000, 1.000000000000000000 ) ) ;
#53557=FACE_OUTER_BOUND ( 'NONE', #68988, .T. ) ;
#53558=EDGE_LOOP ( 'NONE', ( #39508, #78223 ) ) ;
#53559=DIRECTION ( 'NONE',  ( -0.000000000000000000, 1.000000000000000000, -0.000000000000000000 ) ) ;
#53560=EDGE_CURVE ( 'NONE', #103587, #127196, #128306, .T. ) ;
#53561=DIRECTION ( 'NONE',  ( 0.000000000000000000, 0.000000000000000000, 1.000000000000000000 ) ) ;
#53562=CARTESIAN_POINT ( 'NONE',  ( 13.29999999999989946, 2.500000000000000000, -2.385244779468109755E-15 ) ) ;
#53563=ORIENTED_EDGE ( 'NONE', *, *, #18573, .F. ) ;
#53564=EDGE_CURVE ( 'NONE', #64904, #98829, #23754, .T. ) ;
#53565=FACE_OUTER_BOUND ( 'NONE', #57340, .T. ) ;
#53566=ADVANCED_FACE ( 'NONE', ( #128587 ), #113622, .T. ) ;
#53567=CARTESIAN_POINT ( 'NONE',  ( -2.700000000000030376, 2.500000000000000000, 3.883716857408421319 ) ) ;
#53568=ORIENTED_EDGE ( 'NONE', *, *, #32863, .T. ) ;
#53569=AXIS2_PLACEMENT_3D ( 'NONE', #47420, #86685, #35661 ) ;
#53570=VERTEX_POINT ( 'NONE', #118083 ) ;
#53571=ORIENTED_EDGE ( 'NONE', *, *, #112271, .F. ) ;
#53572=ORIENTED_EDGE ( 'NONE', *, *, #30550, .T. ) ;
#53573=PLANE ( 'NONE',  #46831 ) ;
#53574=ADVANCED_FACE ( 'NONE', ( #19228 ), #68344, .T. ) ;
#53575=EDGE_CURVE ( 'NONE', #71342, #45854, #111564, .T. ) ;
#53576=CONICAL_SURFACE ( 'NONE', #87014, 0.1000000000000002554, 0.003490658503988666988 ) ;
#53577=EDGE_CURVE ( 'NONE', #125197, #41184, #69635, .T. ) ;
#53578=VECTOR ( 'NONE', #115237, 1000.000000000000000 ) ;
#53579=EDGE_CURVE ( 'NONE', #31468, #94085, #53231, .T. ) ;
#53580=FACE_OUTER_BOUND ( 'NONE', #24090, .T. ) ;
#53581=DIRECTION ( 'NONE',  ( 0.000000000000000000, 0.000000000000000000, 1.000000000000000000 ) ) ;
#53582=VECTOR ( 'NONE', #32874, 1000.000000000000000 ) ;
#53583=CARTESIAN_POINT ( 'NONE',  ( 13.74999999999989519, 2.500000000000000000, -2.757883832488654097 ) ) ;
#53584=VERTEX_POINT ( 'NONE', #72863 ) ;
#53585=AXIS2_PLACEMENT_3D ( 'NONE', #92912, #53617, #52325 ) ;
#53586=EDGE_CURVE ( 'NONE', #21808, #37517, #120033, .T. ) ;
#53587=FACE_OUTER_BOUND ( 'NONE', #128623, .T. ) ;
#53588=ORIENTED_EDGE ( 'NONE', *, *, #61524, .T. ) ;
#53589=CARTESIAN_POINT ( 'NONE',  ( 4.799999999999934097, 2.500000000000000000, 4.576537180435972019 ) ) ;
#53590=DIRECTION ( 'NONE',  ( 0.000000000000000000, 0.000000000000000000, -1.000000000000000000 ) ) ;
#53591=LINE ( 'NONE', #113139, #21220 ) ;
#53592=CARTESIAN_POINT ( 'NONE',  ( -8.350000000000008527, 12.50000000000000000, 7.188010851410848723 ) ) ;
#53593=ADVANCED_FACE ( 'NONE', ( #70289 ), #86418, .T. ) ;
#53594=CIRCLE ( 'NONE', #49401, 0.1000000000000002554 ) ;
#53595=EDGE_LOOP ( 'NONE', ( #100160, #80928 ) ) ;
#53596=AXIS2_PLACEMENT_3D ( 'NONE', #118371, #39841, #120318 ) ;
#53597=CIRCLE ( 'NONE', #70318, 0.06509327318403741736 ) ;
#53598=VERTEX_POINT ( 'NONE', #110212 ) ;
#53599=VERTEX_POINT ( 'NONE', #40849 ) ;
#53600=DIRECTION ( 'NONE',  ( 0.000000000000000000, 0.000000000000000000, -1.000000000000000000 ) ) ;
#53601=CARTESIAN_POINT ( 'NONE',  ( 6.249999999999968914, 2.500000000000000000, -6.395190528383301931 ) ) ;
#53602=CARTESIAN_POINT ( 'NONE',  ( -11.25000000000000000, 2.500000000000000000, -7.288010851410851032 ) ) ;
#53603=FACE_BOUND ( 'NONE', #87073, .T. ) ;
#53604=CARTESIAN_POINT ( 'NONE',  ( -7.700000000000014388, 2.500000000000000000, -0.4464101615137782142 ) ) ;
#53605=CARTESIAN_POINT ( 'NONE',  ( -14.99999999999998224, 2.500000000000000000, -0.5928203230275518321 ) ) ;
#53606=FACE_OUTER_BOUND ( 'NONE', #60508, .T. ) ;
#53608=FACE_OUTER_BOUND ( 'NONE', #81380, .T. ) ;
#53609=CARTESIAN_POINT ( 'NONE',  ( -4.119968255444916849E-14, 2.500000000000000000, 3.637306695894644726 ) ) ;
#53610=ORIENTED_EDGE ( 'NONE', *, *, #75697, .T. ) ;
#53611=CARTESIAN_POINT ( 'NONE',  ( 10.84999999999991260, 12.50000000000000000, -2.165063509461101710 ) ) ;
#53612=VERTEX_POINT ( 'NONE', #101681 ) ;
#53613=VERTEX_POINT ( 'NONE', #52569 ) ;
#53614=EDGE_LOOP ( 'NONE', ( #97702, #5933, #85277, #53538 ) ) ;
#53615=FACE_OUTER_BOUND ( 'NONE', #65758, .T. ) ;
#53616=FACE_BOUND ( 'NONE', #58344, .T. ) ;
#53617=DIRECTION ( 'NONE',  ( -0.000000000000000000, -1.000000000000000000, -0.000000000000000000 ) ) ;
#53618=AXIS2_PLACEMENT_3D ( 'NONE', #113201, #63476, #113866 ) ;
#53619=EDGE_CURVE ( 'NONE', #6735, #37234, #115669, .T. ) ;
#53621=CARTESIAN_POINT ( 'NONE',  ( -4.400000000000025224, 12.50000000000000000, 4.676537180435972552 ) ) ;
#53622=DIRECTION ( 'NONE',  ( 0.000000000000000000, 0.000000000000000000, -1.000000000000000000 ) ) ;
#53623=VERTEX_POINT ( 'NONE', #61104 ) ;
#53624=PLANE ( 'NONE',  #122234 ) ;
#53625=FACE_OUTER_BOUND ( 'NONE', #124961, .T. ) ;
#53626=AXIS2_PLACEMENT_3D ( 'NONE', #122199, #32545, #16075 ) ;
#53627=EDGE_CURVE ( 'NONE', #52693, #12173, #91213, .T. ) ;
#53628=VERTEX_POINT ( 'NONE', #80107 ) ;
#53629=PLANE ( 'NONE',  #15086 ) ;
#53630=CARTESIAN_POINT ( 'NONE',  ( 12.09999999999990195, 2.500000000000000000, -2.276824562219559311E-15 ) ) ;
#53631=AXIS2_PLACEMENT_3D ( 'NONE', #121796, #92335, #2655 ) ;
#53632=CIRCLE ( 'NONE', #120535, 0.1000000000000002554 ) ;
#53633=ORIENTED_EDGE ( 'NONE', *, *, #51274, .T. ) ;
#53634=AXIS2_PLACEMENT_3D ( 'NONE', #95535, #5836, #85055 ) ;
#53635=DIRECTION ( 'NONE',  ( 0.000000000000000000, 0.000000000000000000, 1.000000000000000000 ) ) ;
#53636=FACE_OUTER_BOUND ( 'NONE', #57500, .T. ) ;
#53637=CARTESIAN_POINT ( 'NONE',  ( -10.20000000000000284, 2.500000000000000000, -0.2464101615137782308 ) ) ;
#53638=ORIENTED_EDGE ( 'NONE', *, *, #48818, .T. ) ;
#53639=ORIENTED_EDGE ( 'NONE', *, *, #102197, .T. ) ;
#53640=LINE ( 'NONE', #4500, #78633 ) ;
#53641=ORIENTED_EDGE ( 'NONE', *, *, #8188, .T. ) ;
#53642=DIRECTION ( 'NONE',  ( 0.000000000000000000, 1.000000000000000000, 0.000000000000000000 ) ) ;
#53643=CARTESIAN_POINT ( 'NONE',  ( -9.600000000000006750, 2.500000000000000000, -0.5928203230275542746 ) ) ;
#53644=ORIENTED_EDGE ( 'NONE', *, *, #107250, .F. ) ;
#53645=DIRECTION ( 'NONE',  ( 0.000000000000000000, 0.000000000000000000, -1.000000000000000000 ) ) ;
#53646=CARTESIAN_POINT ( 'NONE',  ( 9.799999999999915445, 2.500000000000000000, 3.983716857408420964 ) ) ;
#53647=CARTESIAN_POINT ( 'NONE',  ( 4.399999999999940847, 12.50000000000000000, -4.048810130592463530 ) ) ;
#53648=CARTESIAN_POINT ( 'NONE',  ( 4.149999999999941735, 2.500000000000000000, -1.572243186433550211 ) ) ;
#53649=AXIS2_PLACEMENT_3D ( 'NONE', #343, #97271, #109007 ) ;
#53650=CARTESIAN_POINT ( 'NONE',  ( 9.549999999999918998, 2.500000000000000000, -6.495190528383302464 ) ) ;
#53651=VECTOR ( 'NONE', #59125, 1000.000000000000000 ) ;
#53652=ORIENTED_EDGE ( 'NONE', *, *, #13826, .T. ) ;
#53653=EDGE_CURVE ( 'NONE', #105928, #124471, #51942, .T. ) ;
#53654=VERTEX_POINT ( 'NONE', #82025 ) ;
#53655=CARTESIAN_POINT ( 'NONE',  ( -1.250000000000037526, 2.500000000000000000, -1.472243186433550122 ) ) ;
#53656=AXIS2_PLACEMENT_3D ( 'NONE', #128636, #78881, #118781 ) ;
#53658=VERTEX_POINT ( 'NONE', #2174 ) ;
#53659=EDGE_LOOP ( 'NONE', ( #113319, #29613, #4079, #87712 ) ) ;
#53660=ORIENTED_EDGE ( 'NONE', *, *, #96276, .F. ) ;
#53661=CARTESIAN_POINT ( 'NONE',  ( 13.14999999999990088, 2.500000000000000000, 1.918653347947321564 ) ) ;
#53662=AXIS2_PLACEMENT_3D ( 'NONE', #43031, #82936, #33201 ) ;
#53663=AXIS2_PLACEMENT_3D ( 'NONE', #1141, #69890, #48310 ) ;
#53664=FACE_OUTER_BOUND ( 'NONE', #64438, .T. ) ;
#53665=ADVANCED_FACE ( 'NONE', ( #12636 ), #30377, .T. ) ;
#53666=DIRECTION ( 'NONE',  ( 0.000000000000000000, 0.000000000000000000, -1.000000000000000000 ) ) ;
#53667=AXIS2_PLACEMENT_3D ( 'NONE', #89142, #30891, #2041 ) ;
#53668=DIRECTION ( 'NONE',  ( 0.000000000000000000, -0.9999939076577903929, 0.003490651415223739937 ) ) ;
#53669=DIRECTION ( 'NONE',  ( 0.000000000000000000, 0.000000000000000000, 1.000000000000000000 ) ) ;
#53670=DIRECTION ( 'NONE',  ( -0.000000000000000000, 1.000000000000000000, -0.000000000000000000 ) ) ;
#53671=DIRECTION ( 'NONE',  ( 0.000000000000000000, 0.000000000000000000, -1.000000000000000000 ) ) ;
#53672=CARTESIAN_POINT ( 'NONE',  ( 2.499999999999983569, 12.50000000000000000, -4.330127018922201643 ) ) ;
#53673=EDGE_CURVE ( 'NONE', #104031, #126341, #1530, .T. ) ;
#53674=EDGE_CURVE ( 'NONE', #106262, #115994, #100389, .T. ) ;
#53675=CARTESIAN_POINT ( 'NONE',  ( 9.199999999999919353, 12.50000000000000000, -2.276824562219559311E-15 ) ) ;
#53676=VECTOR ( 'NONE', #7379, 1000.000000000000000 ) ;
#53677=VERTEX_POINT ( 'NONE', #72233 ) ;
#53678=AXIS2_PLACEMENT_3D ( 'NONE', #90035, #120162, #40323 ) ;
#53679=AXIS2_PLACEMENT_3D ( 'NONE', #102102, #32737, #3258 ) ;
#53680=EDGE_CURVE ( 'NONE', #129536, #125867, #2812, .T. ) ;
#53681=PLANE ( 'NONE',  #50708 ) ;
#53682=ORIENTED_EDGE ( 'NONE', *, *, #123572, .F. ) ;
#53683=VERTEX_POINT ( 'NONE', #23111 ) ;
#53684=ADVANCED_FACE ( 'NONE', ( #71562 ), #30014, .T. ) ;
#53685=DIRECTION ( 'NONE',  ( 0.000000000000000000, 0.000000000000000000, -1.000000000000000000 ) ) ;
#53686=DIRECTION ( 'NONE',  ( 0.000000000000000000, 0.000000000000000000, 1.000000000000000000 ) ) ;
#53687=FACE_OUTER_BOUND ( 'NONE', #17253, .T. ) ;
#53688=DIRECTION ( 'NONE',  ( 0.000000000000000000, 0.000000000000000000, -1.000000000000000000 ) ) ;
#53689=DIRECTION ( 'NONE',  ( 0.000000000000000000, 0.000000000000000000, 1.000000000000000000 ) ) ;
#53690=FACE_OUTER_BOUND ( 'NONE', #106579, .T. ) ;
#53691=DIRECTION ( 'NONE',  ( -0.000000000000000000, 1.000000000000000000, -0.000000000000000000 ) ) ;
#53692=VERTEX_POINT ( 'NONE', #122611 ) ;
#53693=DIRECTION ( 'NONE',  ( 0.000000000000000000, 0.000000000000000000, -1.000000000000000000 ) ) ;
#53694=TOROIDAL_SURFACE ( 'NONE', #49600, 9.000000000000001776, 1.000000000000000000 ) ;
#53695=CARTESIAN_POINT ( 'NONE',  ( 11.64999999999990798, 2.500000000000000000, -1.572243186433550211 ) ) ;
#53696=VERTEX_POINT ( 'NONE', #32960 ) ;
#53697=ORIENTED_EDGE ( 'NONE', *, *, #39254, .F. ) ;
#53698=ORIENTED_EDGE ( 'NONE', *, *, #26339, .F. ) ;
#53699=ORIENTED_EDGE ( 'NONE', *, *, #71457, .T. ) ;
#53700=DIRECTION ( 'NONE',  ( 0.000000000000000000, -0.9999939076577903929, 0.003490651415223739937 ) ) ;
#53701=CARTESIAN_POINT ( 'NONE',  ( -4.800000000000024691, 12.50000000000000000, 0.3464101615137735735 ) ) ;
#53702=CARTESIAN_POINT ( 'NONE',  ( 1.449999999999952216, 2.500000000000000000, -2.511473670974877948 ) ) ;
#53703=AXIS2_PLACEMENT_3D ( 'NONE', #50051, #39590, #89299 ) ;
#53704=CARTESIAN_POINT ( 'NONE',  ( -1.050000000000038236, 2.500000000000000000, -1.718653347947326049 ) ) ;
#53705=FACE_OUTER_BOUND ( 'NONE', #82470, .T. ) ;
#53706=ORIENTED_EDGE ( 'NONE', *, *, #34811, .T. ) ;
#53707=FACE_OUTER_BOUND ( 'NONE', #27751, .T. ) ;
#53708=CARTESIAN_POINT ( 'NONE',  ( 9.999999999999948486, 12.50000000000000000, -4.265033745738164406 ) ) ;
#53709=LINE ( 'NONE', #33448, #13793 ) ;
#53710=CIRCLE ( 'NONE', #1474, 0.06509327318403745899 ) ;
#53711=AXIS2_PLACEMENT_3D ( 'NONE', #43123, #122313, #31357 ) ;
#53712=CARTESIAN_POINT ( 'NONE',  ( -11.64999999999999680, 2.500000000000000000, 2.857883832488649301 ) ) ;
#53713=ORIENTED_EDGE ( 'NONE', *, *, #68521, .F. ) ;
#53714=ORIENTED_EDGE ( 'NONE', *, *, #46480, .T. ) ;
#53715=ORIENTED_EDGE ( 'NONE', *, *, #3332, .F. ) ;
#53716=ADVANCED_FACE ( 'NONE', ( #112792 ), #69708, .T. ) ;
#53717=DIRECTION ( 'NONE',  ( 0.000000000000000000, 0.000000000000000000, 1.000000000000000000 ) ) ;
#53718=ADVANCED_FACE ( 'NONE', ( #70928 ), #41496, .T. ) ;
#53719=EDGE_CURVE ( 'NONE', #18217, #112183, #9064, .T. ) ;
#53721=CIRCLE ( 'NONE', #28601, 0.1000000000000000472 ) ;
#53722=ADVANCED_FACE ( 'NONE', ( #26347 ), #117802, .T. ) ;
#53723=FACE_OUTER_BOUND ( 'NONE', #53483, .T. ) ;
#53724=DIRECTION ( 'NONE',  ( 0.000000000000000000, 0.000000000000000000, 1.000000000000000000 ) ) ;
#53725=AXIS2_PLACEMENT_3D ( 'NONE', #71651, #72309, #11439 ) ;
#53726=ADVANCED_FACE ( 'NONE', ( #4735 ), #55796, .T. ) ;
#53728=DIRECTION ( 'NONE',  ( 0.000000000000000000, 0.000000000000000000, -1.000000000000000000 ) ) ;
#53729=DIRECTION ( 'NONE',  ( 0.000000000000000000, 0.000000000000000000, 1.000000000000000000 ) ) ;
#53730=CARTESIAN_POINT ( 'NONE',  ( 9.149999999999920419, 12.50000000000000000, -7.253104124594891289 ) ) ;
#53731=CARTESIAN_POINT ( 'NONE',  ( 2.699999999999947331, 2.500000000000000000, -0.2464101615137783419 ) ) ;
#53732=EDGE_CURVE ( 'NONE', #32164, #72823, #25794, .T. ) ;
#53733=EDGE_CURVE ( 'NONE', #29014, #47875, #75957, .T. ) ;
#53734=FACE_OUTER_BOUND ( 'NONE', #48670, .T. ) ;
#53735=EDGE_LOOP ( 'NONE', ( #83863, #119643, #91405, #7430 ) ) ;
#53736=ORIENTED_EDGE ( 'NONE', *, *, #44447, .T. ) ;
#53737=DIRECTION ( 'NONE',  ( -4.274815082592931898E-19, -0.9999939076577903929, -0.003490651415223739937 ) ) ;
#53738=FACE_OUTER_BOUND ( 'NONE', #35057, .T. ) ;
#53739=VECTOR ( 'NONE', #90325, 1000.000000000000000 ) ;
#53740=DIRECTION ( 'NONE',  ( 0.000000000000000000, -0.9999939076577903929, 0.003490651415223739937 ) ) ;
#53741=FACE_OUTER_BOUND ( 'NONE', #93260, .T. ) ;
#53742=AXIS2_PLACEMENT_3D ( 'NONE', #50576, #21115, #61042 ) ;
#53743=CARTESIAN_POINT ( 'NONE',  ( 8.549999999999924327, 2.500000000000000000, 1.818653347947321475 ) ) ;
#53744=EDGE_LOOP ( 'NONE', ( #78101, #29470 ) ) ;
#53745=CIRCLE ( 'NONE', #97661, 0.06509327318403741736 ) ;
#53746=ORIENTED_EDGE ( 'NONE', *, *, #29745, .F. ) ;
#53747=DIRECTION ( 'NONE',  ( 0.000000000000000000, -0.000000000000000000, 1.000000000000000000 ) ) ;
#53748=CARTESIAN_POINT ( 'NONE',  ( -3.100000000000028955, 2.500000000000000000, 3.983716857408420964 ) ) ;
#53749=AXIS2_PLACEMENT_3D ( 'NONE', #80848, #31116, #9524 ) ;
#53750=CARTESIAN_POINT ( 'NONE',  ( -10.84999999999999964, 2.500000000000000000, 1.472243186433545459 ) ) ;
#53751=AXIS2_PLACEMENT_3D ( 'NONE', #6274, #114947, #4992 ) ;
#53752=DIRECTION ( 'NONE',  ( 0.000000000000000000, 0.000000000000000000, 1.000000000000000000 ) ) ;
#53753=ORIENTED_EDGE ( 'NONE', *, *, #59657, .T. ) ;
#53754=CARTESIAN_POINT ( 'NONE',  ( 10.44999999999991402, 2.500000000000000000, 6.495190528383297135 ) ) ;
#53755=CIRCLE ( 'NONE', #126928, 0.1000000000000002554 ) ;
#53756=DIRECTION ( 'NONE',  ( 0.000000000000000000, 0.000000000000000000, 1.000000000000000000 ) ) ;
#53757=ORIENTED_EDGE ( 'NONE', *, *, #127280, .T. ) ;
#53758=DIRECTION ( 'NONE',  ( 0.000000000000000000, 0.000000000000000000, 1.000000000000000000 ) ) ;
#53759=ORIENTED_EDGE ( 'NONE', *, *, #55932, .F. ) ;
#53760=DIRECTION ( 'NONE',  ( 0.000000000000000000, 1.000000000000000000, 0.000000000000000000 ) ) ;
#53761=AXIS2_PLACEMENT_3D ( 'NONE', #105678, #25825, #76863 ) ;
#53762=AXIS2_PLACEMENT_3D ( 'NONE', #96926, #110460, #98216 ) ;
#53763=ORIENTED_EDGE ( 'NONE', *, *, #46005, .T. ) ;
#53764=CARTESIAN_POINT ( 'NONE',  ( 14.34999999999989306, 2.500000000000000000, -2.411473670974877859 ) ) ;
#53765=DIRECTION ( 'NONE',  ( 0.000000000000000000, 0.000000000000000000, -1.000000000000000000 ) ) ;
#53766=EDGE_LOOP ( 'NONE', ( #19112, #61300 ) ) ;
#53767=VERTEX_POINT ( 'NONE', #74152 ) ;
#53769=LINE ( 'NONE', #112055, #85337 ) ;
#53772=ADVANCED_FACE ( 'NONE', ( #45989 ), #124081, .T. ) ;
#53774=CARTESIAN_POINT ( 'NONE',  ( 5.799999999999931433, 12.50000000000000000, 4.330127018922196314 ) ) ;
#53775=DIRECTION ( 'NONE',  ( 0.000000000000000000, 0.000000000000000000, 1.000000000000000000 ) ) ;
#53776=DIRECTION ( 'NONE',  ( -0.000000000000000000, 1.000000000000000000, -0.000000000000000000 ) ) ;
#53777=AXIS2_PLACEMENT_3D ( 'NONE', #116046, #87857, #66927 ) ;
#53778=ORIENTED_EDGE ( 'NONE', *, *, #60831, .F. ) ;
#53779=ORIENTED_EDGE ( 'NONE', *, *, #110090, .T. ) ;
#53780=CARTESIAN_POINT ( 'NONE',  ( -8.350000000000010303, 2.500000000000000000, 6.495190528383297135 ) ) ;
#53781=VERTEX_POINT ( 'NONE', #55158 ) ;
#53782=DIRECTION ( 'NONE',  ( -0.000000000000000000, 1.000000000000000000, -0.000000000000000000 ) ) ;
#53783=DIRECTION ( 'NONE',  ( 0.000000000000000000, -0.000000000000000000, 1.000000000000000000 ) ) ;
#53785=EDGE_LOOP ( 'NONE', ( #120248, #84247 ) ) ;
#53786=ORIENTED_EDGE ( 'NONE', *, *, #22712, .T. ) ;
#53787=CARTESIAN_POINT ( 'NONE',  ( -3.350000000000028511, 12.50000000000000000, 1.472243186433545459 ) ) ;
#53788=ORIENTED_EDGE ( 'NONE', *, *, #70358, .F. ) ;
#53789=DIRECTION ( 'NONE',  ( 0.000000000000000000, 1.000000000000000000, 0.000000000000000000 ) ) ;
#53791=ORIENTED_EDGE ( 'NONE', *, *, #70120, .F. ) ;
#53792=LINE ( 'NONE', #24344, #7372 ) ;
#53793=CARTESIAN_POINT ( 'NONE',  ( 7.899999999999921307, 12.50000000000000000, -2.385244779468109755E-15 ) ) ;
#53794=AXIS2_PLACEMENT_3D ( 'NONE', #67659, #59820, #78801 ) ;
#53795=DIRECTION ( 'NONE',  ( 0.000000000000000000, 1.000000000000000000, 0.000000000000000000 ) ) ;
#53796=CONICAL_SURFACE ( 'NONE', #49708, 0.1000000000000002554, 0.003490658503988666988 ) ;
#53797=CARTESIAN_POINT ( 'NONE',  ( 9.999999999999914735, 12.50000000000000000, 0.6928203230275494784 ) ) ;
#53798=DIRECTION ( 'NONE',  ( 0.000000000000000000, 0.000000000000000000, 1.000000000000000000 ) ) ;
#53799=CARTESIAN_POINT ( 'NONE',  ( 15.39999999999989022, 2.500000000000000000, -2.385244779468109755E-15 ) ) ;
#53801=DIRECTION ( 'NONE',  ( -0.000000000000000000, 1.000000000000000000, -0.000000000000000000 ) ) ;
#53802=CARTESIAN_POINT ( 'NONE',  ( -7.100000000000017408, 12.50000000000000000, -5.088040615133791356 ) ) ;
#53803=AXIS2_PLACEMENT_3D ( 'NONE', #86895, #37802, #96073 ) ;
#53804=VECTOR ( 'NONE', #576, 1000.000000000000000 ) ;
#53805=VERTEX_POINT ( 'NONE', #104876 ) ;
#53806=VERTEX_POINT ( 'NONE', #85879 ) ;
#53807=CIRCLE ( 'NONE', #126975, 0.06509327318403745899 ) ;
#53808=ORIENTED_EDGE ( 'NONE', *, *, #16067, .F. ) ;
#53809=DIRECTION ( 'NONE',  ( -0.000000000000000000, -1.000000000000000000, -0.000000000000000000 ) ) ;
#53810=VERTEX_POINT ( 'NONE', #36168 ) ;
#53811=ORIENTED_EDGE ( 'NONE', *, *, #42527, .T. ) ;
#53812=ORIENTED_EDGE ( 'NONE', *, *, #121679, .F. ) ;
#53813=ORIENTED_EDGE ( 'NONE', *, *, #86763, .T. ) ;
#53814=EDGE_CURVE ( 'NONE', #29011, #7017, #55139, .T. ) ;
#53815=CARTESIAN_POINT ( 'NONE',  ( 13.09999999999990195, 12.50000000000000000, 3.983716857408420076 ) ) ;
#53816=CIRCLE ( 'NONE', #87248, 0.1000000000000002554 ) ;
#53817=CONICAL_SURFACE ( 'NONE', #26356, 0.1000000000000002554, 0.003490658503988666988 ) ;
#53818=AXIS2_PLACEMENT_3D ( 'NONE', #114005, #43981, #83880 ) ;
#53819=EDGE_CURVE ( 'NONE', #21551, #116826, #94840, .T. ) ;
#53820=DIRECTION ( 'NONE',  ( 0.000000000000000000, 0.000000000000000000, -1.000000000000000000 ) ) ;
#53821=CARTESIAN_POINT ( 'NONE',  ( -5.850000000000021849, 12.50000000000000000, -2.922977105672691422 ) ) ;
#53822=CARTESIAN_POINT ( 'NONE',  ( 13.74999999999993072, 2.500000000000000000, -2.065063509461102065 ) ) ;
#53823=DIRECTION ( 'NONE',  ( 0.000000000000000000, 0.000000000000000000, 1.000000000000000000 ) ) ;
#53824=EDGE_CURVE ( 'NONE', #123556, #92862, #13261, .T. ) ;
#53825=ORIENTED_EDGE ( 'NONE', *, *, #35579, .T. ) ;
#53826=ADVANCED_FACE ( 'NONE', ( #35524 ), #84374, .T. ) ;
#53827=DIRECTION ( 'NONE',  ( -0.000000000000000000, -1.000000000000000000, -0.000000000000000000 ) ) ;
#53829=VECTOR ( 'NONE', #103047, 1000.000000000000000 ) ;
#53830=ORIENTED_EDGE ( 'NONE', *, *, #49233, .F. ) ;
#53831=EDGE_LOOP ( 'NONE', ( #37405, #101110, #108412, #72286 ) ) ;
#53832=CONICAL_SURFACE ( 'NONE', #7844, 0.1000000000000000472, 0.003490658503988666988 ) ;
#53833=ADVANCED_FACE ( 'NONE', ( #16494 ), #61410, .T. ) ;
#53834=DIRECTION ( 'NONE',  ( 0.000000000000000000, 1.000000000000000000, 0.000000000000000000 ) ) ;
#53835=EDGE_CURVE ( 'NONE', #18676, #50283, #78130, .T. ) ;
#53836=EDGE_CURVE ( 'NONE', #75250, #100878, #64958, .T. ) ;
#53837=ORIENTED_EDGE ( 'NONE', *, *, #90994, .T. ) ;
#53838=ORIENTED_EDGE ( 'NONE', *, *, #34157, .F. ) ;
#53839=ADVANCED_FACE ( 'NONE', ( #74800 ), #93797, .T. ) ;
#53840=EDGE_CURVE ( 'NONE', #72027, #99397, #90418, .T. ) ;
#53842=VECTOR ( 'NONE', #41761, 1000.000000000000000 ) ;
#53843=CIRCLE ( 'NONE', #66349, 0.1000000000000002554 ) ;
#53844=CARTESIAN_POINT ( 'NONE',  ( -11.84999999999999609, 2.500000000000000000, 2.511473670974873507 ) ) ;
#53845=CARTESIAN_POINT ( 'NONE',  ( -9.550000000000002487, 12.50000000000000000, 6.495190528383297135 ) ) ;
#53846=DIRECTION ( 'NONE',  ( 0.000000000000000000, 0.000000000000000000, 1.000000000000000000 ) ) ;
#53847=AXIS2_PLACEMENT_3D ( 'NONE', #97194, #10103, #109600 ) ;
#53848=CARTESIAN_POINT ( 'NONE',  ( -6.850000000000017408, 12.50000000000000000, -2.511473670974877948 ) ) ;
#53849=FACE_OUTER_BOUND ( 'NONE', #115873, .T. ) ;
#53850=DIRECTION ( 'NONE',  ( 0.000000000000000000, 0.000000000000000000, -1.000000000000000000 ) ) ;
#53851=ADVANCED_FACE ( 'NONE', ( #25682 ), #99055, .T. ) ;
#53852=CONICAL_SURFACE ( 'NONE', #118683, 0.09999999999999982514, 0.003490658503988666988 ) ;
#53853=DIRECTION ( 'NONE',  ( -0.000000000000000000, 1.000000000000000000, -0.000000000000000000 ) ) ;
#53854=AXIS2_PLACEMENT_3D ( 'NONE', #18690, #99204, #88047 ) ;
#53855=ORIENTED_EDGE ( 'NONE', *, *, #33783, .T. ) ;
#53856=AXIS2_PLACEMENT_3D ( 'NONE', #126306, #36653, #85082 ) ;
#53857=AXIS2_PLACEMENT_3D ( 'NONE', #113284, #93020, #3342 ) ;
#53858=LINE ( 'NONE', #4094, #94493 ) ;
#53859=EDGE_LOOP ( 'NONE', ( #68836, #45688, #6804, #32591 ) ) ;
#53860=CARTESIAN_POINT ( 'NONE',  ( 3.749999999999975131, 2.500000000000000000, 6.495190528383297135 ) ) ;
#53861=EDGE_LOOP ( 'NONE', ( #78233, #17693, #72248, #65229 ) ) ;
#53862=CIRCLE ( 'NONE', #97772, 0.1000000000000000472 ) ;
#53863=ORIENTED_EDGE ( 'NONE', *, *, #127186, .F. ) ;
#53864=CARTESIAN_POINT ( 'NONE',  ( 9.999999999999916511, 2.500000000000000000, -0.6928203230275541413 ) ) ;
#53865=CARTESIAN_POINT ( 'NONE',  ( -8.550000000000013145, 2.500000000000000000, -1.918653347947326004 ) ) ;
#53866=CIRCLE ( 'NONE', #106192, 0.09999999999999982514 ) ;
#53867=CIRCLE ( 'NONE', #127034, 0.09999999999999982514 ) ;
#53868=DIRECTION ( 'NONE',  ( -4.274815082592931898E-19, -0.9999939076577903929, -0.003490651415223739937 ) ) ;
#53869=VERTEX_POINT ( 'NONE', #54496 ) ;
#53870=ORIENTED_EDGE ( 'NONE', *, *, #81842, .T. ) ;
#53871=DIRECTION ( 'NONE',  ( 0.000000000000000000, -0.9999939076577903929, 0.003490651415223739937 ) ) ;
#53872=DIRECTION ( 'NONE',  ( 0.000000000000000000, 1.000000000000000000, 0.000000000000000000 ) ) ;
#53874=CARTESIAN_POINT ( 'NONE',  ( 12.09999999999990195, 2.500000000000000000, -0.1000000000000022815 ) ) ;
#53875=PLANE ( 'NONE',  #68089 ) ;
#53876=CARTESIAN_POINT ( 'NONE',  ( 6.649999999999931966, 12.50000000000000000, -7.188010851410854052 ) ) ;
#53878=EDGE_CURVE ( 'NONE', #112383, #43675, #113432, .T. ) ;
#53879=AXIS2_PLACEMENT_3D ( 'NONE', #8382, #117675, #89532 ) ;
#53880=EDGE_CURVE ( 'NONE', #51819, #11852, #59691, .T. ) ;
#53881=ORIENTED_EDGE ( 'NONE', *, *, #103649, .F. ) ;
#53882=DIRECTION ( 'NONE',  ( -0.000000000000000000, 1.000000000000000000, -0.000000000000000000 ) ) ;
#53883=DIRECTION ( 'NONE',  ( 0.000000000000000000, 0.000000000000000000, -1.000000000000000000 ) ) ;
#53884=EDGE_CURVE ( 'NONE', #120135, #107678, #75763, .T. ) ;
#53886=CARTESIAN_POINT ( 'NONE',  ( 9.799999999999915445, 12.50000000000000000, -4.741630453620015118 ) ) ;
#53887=CARTESIAN_POINT ( 'NONE',  ( -6.700000000000019718, 12.50000000000000000, -4.330127018922201643 ) ) ;
#53888=EDGE_CURVE ( 'NONE', #99960, #74427, #97650, .T. ) ;
#53889=DIRECTION ( 'NONE',  ( 0.000000000000000000, 1.000000000000000000, 0.000000000000000000 ) ) ;
#53890=CARTESIAN_POINT ( 'NONE',  ( 3.949999999999941558, 2.500000000000000000, -6.248780366869526759 ) ) ;
#53891=ORIENTED_EDGE ( 'NONE', *, *, #122610, .T. ) ;
#53892=EDGE_CURVE ( 'NONE', #32647, #46243, #58392, .T. ) ;
#53893=AXIS2_PLACEMENT_3D ( 'NONE', #125151, #75387, #35491 ) ;
#53894=ADVANCED_FACE ( 'NONE', ( #48561 ), #107473, .T. ) ;
#53895=DIRECTION ( 'NONE',  ( -0.000000000000000000, 1.000000000000000000, -0.000000000000000000 ) ) ;
#53896=CIRCLE ( 'NONE', #10074, 0.06509327318403745899 ) ;
#53897=ADVANCED_FACE ( 'NONE', ( #46613 ), #2909, .T. ) ;
#53898=DIRECTION ( 'NONE',  ( 0.000000000000000000, 1.000000000000000000, 0.000000000000000000 ) ) ;
#53899=CARTESIAN_POINT ( 'NONE',  ( -8.950000000000008171, 12.50000000000000000, 1.818653347947321475 ) ) ;
#53900=ORIENTED_EDGE ( 'NONE', *, *, #75461, .T. ) ;
#53901=EDGE_CURVE ( 'NONE', #82923, #81743, #109517, .T. ) ;
#53902=FACE_OUTER_BOUND ( 'NONE', #3358, .T. ) ;
#53903=VECTOR ( 'NONE', #32118, 1000.000000000000000 ) ;
#53904=AXIS2_PLACEMENT_3D ( 'NONE', #110793, #21123, #11306 ) ;
#53905=ORIENTED_EDGE ( 'NONE', *, *, #110974, .F. ) ;
#53906=DIRECTION ( 'NONE',  ( 0.000000000000000000, 0.000000000000000000, 1.000000000000000000 ) ) ;
#53907=ORIENTED_EDGE ( 'NONE', *, *, #79715, .F. ) ;
#53908=CARTESIAN_POINT ( 'NONE',  ( -2.950000000000029932, 12.50000000000000000, -2.165063509461101710 ) ) ;
#53909=CARTESIAN_POINT ( 'NONE',  ( -11.84999999999999609, 2.500000000000000000, 6.248780366869521430 ) ) ;
#53910=DIRECTION ( 'NONE',  ( -0.000000000000000000, 1.000000000000000000, -0.000000000000000000 ) ) ;
#53911=ORIENTED_EDGE ( 'NONE', *, *, #66107, .T. ) ;
#53912=VECTOR ( 'NONE', #111912, 1000.000000000000000 ) ;
#53913=DIRECTION ( 'NONE',  ( 0.000000000000000000, 0.000000000000000000, 1.000000000000000000 ) ) ;
#53914=CARTESIAN_POINT ( 'NONE',  ( -4.600000000000028066, 2.500000000000000000, -3.637306695894650055 ) ) ;
#53915=CIRCLE ( 'NONE', #68574, 0.06509327318403745899 ) ;
#53916=ADVANCED_FACE ( 'NONE', ( #57070 ), #88461, .T. ) ;
#53917=ORIENTED_EDGE ( 'NONE', *, *, #7943, .F. ) ;
#53918=CARTESIAN_POINT ( 'NONE',  ( 9.349999999999919709, 2.500000000000000000, 2.411473670974873862 ) ) ;
#53919=CIRCLE ( 'NONE', #127094, 0.06509327318403745899 ) ;
#53920=EDGE_LOOP ( 'NONE', ( #78800, #125918 ) ) ;
#53921=ORIENTED_EDGE ( 'NONE', *, *, #15385, .F. ) ;
#53922=AXIS2_PLACEMENT_3D ( 'NONE', #117372, #110174, #20507 ) ;
#53923=CARTESIAN_POINT ( 'NONE',  ( 1.899999999999949507, 2.500000000000000000, 4.776537180435972196 ) ) ;
#53924=CARTESIAN_POINT ( 'NONE',  ( -8.750000000000012434, 12.50000000000000000, -5.737276932171707422 ) ) ;
#53926=ORIENTED_EDGE ( 'NONE', *, *, #76141, .T. ) ;
#53927=AXIS2_PLACEMENT_3D ( 'NONE', #123219, #44018, #74120 ) ;
#53928=DIRECTION ( 'NONE',  ( 0.000000000000000000, 0.000000000000000000, 1.000000000000000000 ) ) ;
#53929=CARTESIAN_POINT ( 'NONE',  ( -1.650000000000035660, 12.50000000000000000, 2.792790559304612064 ) ) ;
#53930=VECTOR ( 'NONE', #95532, 1000.000000000000000 ) ;
#53931=EDGE_LOOP ( 'NONE', ( #82924, #99578 ) ) ;
#53932=CARTESIAN_POINT ( 'NONE',  ( -4.150000000000027889, 2.500000000000000000, -6.495190528383302464 ) ) ;
#53933=DIRECTION ( 'NONE',  ( 0.000000000000000000, 0.000000000000000000, 1.000000000000000000 ) ) ;
#53934=AXIS2_PLACEMENT_3D ( 'NONE', #31058, #121997, #100420 ) ;
#53935=ADVANCED_FACE ( 'NONE', ( #47277 ), #17251, .T. ) ;
#53936=CARTESIAN_POINT ( 'NONE',  ( -13.74999999999998934, 12.50000000000000000, 2.792790559304615616 ) ) ;
#53937=FACE_OUTER_BOUND ( 'NONE', #96244, .T. ) ;
#53938=PLANE ( 'NONE',  #101045 ) ;
#53939=DIRECTION ( 'NONE',  ( 0.000000000000000000, 1.000000000000000000, 0.000000000000000000 ) ) ;
#53940=AXIS2_PLACEMENT_3D ( 'NONE', #105486, #6593, #36104 ) ;
#53941=DIRECTION ( 'NONE',  ( 0.000000000000000000, 1.000000000000000000, 0.000000000000000000 ) ) ;
#53942=AXIS2_PLACEMENT_3D ( 'NONE', #70231, #57177, #48020 ) ;
#53943=AXIS2_PLACEMENT_3D ( 'NONE', #82418, #122970, #53590 ) ;
#53944=ORIENTED_EDGE ( 'NONE', *, *, #7632, .T. ) ;
#53945=ORIENTED_EDGE ( 'NONE', *, *, #117507, .F. ) ;
#53946=ORIENTED_EDGE ( 'NONE', *, *, #31132, .F. ) ;
#53947=ORIENTED_EDGE ( 'NONE', *, *, #65784, .T. ) ;
#53948=FACE_OUTER_BOUND ( 'NONE', #32877, .T. ) ;
#53949=CARTESIAN_POINT ( 'NONE',  ( -3.350000000000031619, 2.500000000000000000, -7.188010851410854052 ) ) ;
#53950=CARTESIAN_POINT ( 'NONE',  ( -1.250000000000036193, 2.500000000000000000, 5.702370205355745014 ) ) ;
#53951=VERTEX_POINT ( 'NONE', #27602 ) ;
#53952=ADVANCED_FACE ( 'NONE', ( #67521 ), #7973, .T. ) ;
#53953=FACE_BOUND ( 'NONE', #14957, .T. ) ;
#53954=FACE_OUTER_BOUND ( 'NONE', #10938, .T. ) ;
#53955=DIRECTION ( 'NONE',  ( 0.000000000000000000, 1.000000000000000000, 0.000000000000000000 ) ) ;
#53956=DIRECTION ( 'NONE',  ( -0.000000000000000000, 1.000000000000000000, -0.000000000000000000 ) ) ;
#53957=AXIS2_PLACEMENT_3D ( 'NONE', #72535, #34555, #64628 ) ;
#53958=AXIS2_PLACEMENT_3D ( 'NONE', #12516, #103492, #13798 ) ;
#53959=CARTESIAN_POINT ( 'NONE',  ( 12.04999999999990834, 2.500000000000000000, -2.165063509461101710 ) ) ;
#53960=LINE ( 'NONE', #53327, #122485 ) ;
#53961=CARTESIAN_POINT ( 'NONE',  ( -3.950000000000024603, 12.50000000000000000, 1.818653347947321475 ) ) ;
#53962=CARTESIAN_POINT ( 'NONE',  ( -6.050000000000018474, 12.50000000000000000, 6.906693963081109722 ) ) ;
#53963=FACE_OUTER_BOUND ( 'NONE', #38201, .T. ) ;
#53965=DIRECTION ( 'NONE',  ( 0.000000000000000000, -0.000000000000000000, 1.000000000000000000 ) ) ;
#53966=ORIENTED_EDGE ( 'NONE', *, *, #58146, .F. ) ;
#53967=ORIENTED_EDGE ( 'NONE', *, *, #106937, .T. ) ;
#53968=ORIENTED_EDGE ( 'NONE', *, *, #89947, .T. ) ;
#53969=ORIENTED_EDGE ( 'NONE', *, *, #109065, .F. ) ;
#53970=EDGE_LOOP ( 'NONE', ( #97881, #80517 ) ) ;
#53971=ORIENTED_EDGE ( 'NONE', *, *, #101129, .T. ) ;
#53972=CARTESIAN_POINT ( 'NONE',  ( -10.65000000000000213, 2.500000000000000000, 1.818653347947321475 ) ) ;
#53973=VERTEX_POINT ( 'NONE', #86539 ) ;
#53974=ORIENTED_EDGE ( 'NONE', *, *, #42544, .F. ) ;
#53975=ADVANCED_FACE ( 'NONE', ( #116641 ), #48895, .T. ) ;
#53976=CARTESIAN_POINT ( 'NONE',  ( 12.31005523291632464, -2.500000000000000444, 7.488833080795306962 ) ) ;
#53977=AXIS2_PLACEMENT_3D ( 'NONE', #53646, #124323, #74576 ) ;
#53978=CIRCLE ( 'NONE', #24733, 0.1000000000000002554 ) ;
#53979=DIRECTION ( 'NONE',  ( 0.000000000000000000, 0.000000000000000000, 1.000000000000000000 ) ) ;
#53980=CARTESIAN_POINT ( 'NONE',  ( -3.350000000000028511, 2.500000000000000000, -2.857883832488653741 ) ) ;
#53981=CIRCLE ( 'NONE', #93685, 0.1000000000000000056 ) ;
#53982=EDGE_LOOP ( 'NONE', ( #118243, #10087 ) ) ;
#53983=CARTESIAN_POINT ( 'NONE',  ( 10.39999999999991154, 2.500000000000000000, -5.122947341949753763 ) ) ;
#53984=ADVANCED_FACE ( 'NONE', ( #47923 ), #82336, .T. ) ;
#53985=CONICAL_SURFACE ( 'NONE', #87418, 0.1000000000000002554, 0.003490658503988666988 ) ;
#53986=ORIENTED_EDGE ( 'NONE', *, *, #109915, .T. ) ;
#53987=CONICAL_SURFACE ( 'NONE', #127156, 0.09999999999999982514, 0.003490658503988666988 ) ;
#53988=ORIENTED_EDGE ( 'NONE', *, *, #74978, .F. ) ;
#53989=CARTESIAN_POINT ( 'NONE',  ( -1.650000000000034328, 2.500000000000000000, -6.595190528383302109 ) ) ;
#53990=VERTEX_POINT ( 'NONE', #89122 ) ;
#53991=EDGE_CURVE ( 'NONE', #62914, #2669, #7325, .T. ) ;
#53992=CARTESIAN_POINT ( 'NONE',  ( -9.200000000000006395, 12.50000000000000000, 4.395220292106234439 ) ) ;
#53993=EDGE_CURVE ( 'NONE', #119558, #47762, #108111, .T. ) ;
#53994=ADVANCED_FACE ( 'NONE', ( #117927 ), #76067, .T. ) ;
#53995=EDGE_CURVE ( 'NONE', #85395, #74962, #107154, .T. ) ;
#53996=VERTEX_POINT ( 'NONE', #129073 ) ;
#53997=AXIS2_PLACEMENT_3D ( 'NONE', #75792, #5750, #106546 ) ;
#53998=DIRECTION ( 'NONE',  ( 0.000000000000000000, 1.000000000000000000, 0.000000000000000000 ) ) ;
#53999=AXIS2_PLACEMENT_3D ( 'NONE', #81126, #23480, #121674 ) ;
#54000=DIRECTION ( 'NONE',  ( 0.000000000000000000, -0.9999939076577903929, 0.003490651415223739937 ) ) ;
#54001=LINE ( 'NONE', #73620, #1873 ) ;
#54002=DIRECTION ( 'NONE',  ( -0.000000000000000000, 1.000000000000000000, -0.000000000000000000 ) ) ;
#54003=DIRECTION ( 'NONE',  ( 0.000000000000000000, -0.9999939076577903929, 0.003490651415223739937 ) ) ;
#54004=ADVANCED_FACE ( 'NONE', ( #39407 ), #42638, .T. ) ;
#54005=ORIENTED_EDGE ( 'NONE', *, *, #128959, .F. ) ;
#54006=CARTESIAN_POINT ( 'NONE',  ( 0.3999999999999563904, 2.500000000000000000, 3.537306695894645081 ) ) ;
#54007=EDGE_CURVE ( 'NONE', #1863, #81765, #120520, .T. ) ;
#54008=CIRCLE ( 'NONE', #112501, 0.1000000000000000056 ) ;
#54009=ADVANCED_FACE ( 'NONE', ( #22332 ), #50736, .T. ) ;
#54010=VERTEX_POINT ( 'NONE', #20386 ) ;
#54011=CARTESIAN_POINT ( 'NONE',  ( 87.50000000000004263, 7.402262750143062675, 1.385127402881716874 ) ) ;
#54012=EDGE_LOOP ( 'NONE', ( #45820, #51087, #105751, #34090 ) ) ;
#54013=CARTESIAN_POINT ( 'NONE',  ( -0.8500000000000386136, 2.500000000000000000, 1.572243186433545548 ) ) ;
#54014=DIRECTION ( 'NONE',  ( 0.000000000000000000, 1.000000000000000000, 0.000000000000000000 ) ) ;
#54015=AXIS2_PLACEMENT_3D ( 'NONE', #33594, #45993, #23773 ) ;
#54016=DIRECTION ( 'NONE',  ( 0.000000000000000000, 1.000000000000000000, 0.000000000000000000 ) ) ;
#54017=DIRECTION ( 'NONE',  ( 0.000000000000000000, -0.9999939076577903929, 0.003490651415223739937 ) ) ;
#54018=ORIENTED_EDGE ( 'NONE', *, *, #39384, .T. ) ;
#54021=CARTESIAN_POINT ( 'NONE',  ( -5.650000000000023448, 2.500000000000000000, -2.411473670974877859 ) ) ;
#54022=ORIENTED_EDGE ( 'NONE', *, *, #115399, .F. ) ;
#54023=ORIENTED_EDGE ( 'NONE', *, *, #35094, .F. ) ;
#54024=ORIENTED_EDGE ( 'NONE', *, *, #14547, .F. ) ;
#54025=DIRECTION ( 'NONE',  ( -0.000000000000000000, 1.000000000000000000, -0.000000000000000000 ) ) ;
#54026=DIRECTION ( 'NONE',  ( -0.000000000000000000, 1.000000000000000000, -0.000000000000000000 ) ) ;
#54028=DIRECTION ( 'NONE',  ( 0.000000000000000000, 1.000000000000000000, 0.000000000000000000 ) ) ;
#54029=AXIS2_PLACEMENT_3D ( 'NONE', #26782, #106624, #96797 ) ;
#54030=AXIS2_PLACEMENT_3D ( 'NONE', #41989, #70164, #2045 ) ;
#54031=DIRECTION ( 'NONE',  ( 0.000000000000000000, 0.000000000000000000, -1.000000000000000000 ) ) ;
#54032=CARTESIAN_POINT ( 'NONE',  ( -3.550000000000028244, 2.500000000000000000, -1.918653347947326004 ) ) ;
#54033=VECTOR ( 'NONE', #54429, 1000.000000000000000 ) ;
#54034=ORIENTED_EDGE ( 'NONE', *, *, #19830, .F. ) ;
#54035=FACE_OUTER_BOUND ( 'NONE', #59237, .T. ) ;
#54036=ORIENTED_EDGE ( 'NONE', *, *, #30343, .F. ) ;
#54037=DIRECTION ( 'NONE',  ( -0.000000000000000000, 1.000000000000000000, -0.000000000000000000 ) ) ;
#54038=VECTOR ( 'NONE', #90139, 1000.000000000000000 ) ;
#54039=DIRECTION ( 'NONE',  ( 0.000000000000000000, 1.000000000000000000, 0.000000000000000000 ) ) ;
#54041=ADVANCED_FACE ( 'NONE', ( #11191 ), #46514, .T. ) ;
#54042=CARTESIAN_POINT ( 'NONE',  ( -9.200000000000006395, 2.500000000000000000, -0.1000000000000023925 ) ) ;
#54043=ORIENTED_EDGE ( 'NONE', *, *, #56811, .F. ) ;
#54044=EDGE_CURVE ( 'NONE', #79461, #100575, #41332, .T. ) ;
#54045=VECTOR ( 'NONE', #112228, 1000.000000000000000 ) ;
#54046=AXIS2_PLACEMENT_3D ( 'NONE', #7674, #55510, #66604 ) ;
#54047=ADVANCED_FACE ( 'NONE', ( #112636 ), #122040, .T. ) ;
#54048=FACE_OUTER_BOUND ( 'NONE', #27122, .T. ) ;
#54049=DIRECTION ( 'NONE',  ( -0.000000000000000000, 1.000000000000000000, -0.000000000000000000 ) ) ;
#54050=EDGE_LOOP ( 'NONE', ( #125796, #107489, #60999, #73207 ) ) ;
#54052=EDGE_CURVE ( 'NONE', #112102, #7001, #12487, .T. ) ;
#54053=DIRECTION ( 'NONE',  ( 0.000000000000000000, 1.000000000000000000, 0.000000000000000000 ) ) ;
#54054=VERTEX_POINT ( 'NONE', #71393 ) ;
#54055=EDGE_LOOP ( 'NONE', ( #45617, #10031 ) ) ;
#54056=CARTESIAN_POINT ( 'NONE',  ( -0.2000000000000404232, 12.50000000000000000, 4.048810130592458201 ) ) ;
#54057=CIRCLE ( 'NONE', #14324, 0.06509327318403745899 ) ;
#54058=ORIENTED_EDGE ( 'NONE', *, *, #115917, .F. ) ;
#54059=LINE ( 'NONE', #44894, #94876 ) ;
#54060=CARTESIAN_POINT ( 'NONE',  ( -13.14999999999999147, 2.500000000000000000, 1.718653347947325383 ) ) ;
#54061=DIRECTION ( 'NONE',  ( 0.000000000000000000, 0.000000000000000000, 1.000000000000000000 ) ) ;
#54063=VECTOR ( 'NONE', #90556, 1000.000000000000000 ) ;
#54064=AXIS2_PLACEMENT_3D ( 'NONE', #128880, #107915, #39209 ) ;
#54065=CARTESIAN_POINT ( 'NONE',  ( 13.29999999999990301, 12.50000000000000000, 4.330127018922196314 ) ) ;
#54066=DIRECTION ( 'NONE',  ( -4.274815082592931898E-19, -0.9999939076577903929, -0.003490651415223739937 ) ) ;
#54067=ORIENTED_EDGE ( 'NONE', *, *, #110729, .T. ) ;
#54068=FACE_OUTER_BOUND ( 'NONE', #34827, .T. ) ;
#54069=FACE_OUTER_BOUND ( 'NONE', #119399, .T. ) ;
#54070=EDGE_CURVE ( 'NONE', #105674, #50587, #63550, .T. ) ;
#54071=AXIS2_PLACEMENT_3D ( 'NONE', #124498, #84565, #34844 ) ;
#54072=ORIENTED_EDGE ( 'NONE', *, *, #44362, .T. ) ;
#54073=AXIS2_PLACEMENT_3D ( 'NONE', #109371, #39374, #27570 ) ;
#54074=CIRCLE ( 'NONE', #47829, 0.1000000000000000472 ) ;
#54075=EDGE_LOOP ( 'NONE', ( #39576, #41320 ) ) ;
#54076=CONICAL_SURFACE ( 'NONE', #26889, 0.1000000000000000472, 0.003490658503988666988 ) ;
#54077=VERTEX_POINT ( 'NONE', #100236 ) ;
#54078=DIRECTION ( 'NONE',  ( 0.000000000000000000, 0.000000000000000000, -1.000000000000000000 ) ) ;
#54079=DIRECTION ( 'NONE',  ( 0.000000000000000000, 0.000000000000000000, 1.000000000000000000 ) ) ;
#54080=CARTESIAN_POINT ( 'NONE',  ( 9.399999999999915090, 2.500000000000000000, -4.776537180435977525 ) ) ;
#54081=FACE_BOUND ( 'NONE', #10049, .T. ) ;
#54082=ORIENTED_EDGE ( 'NONE', *, *, #35980, .T. ) ;
#54084=CONICAL_SURFACE ( 'NONE', #18580, 0.09999999999999982514, 0.003490658503988666988 ) ;
#54085=DIRECTION ( 'NONE',  ( 0.000000000000000000, 0.000000000000000000, -1.000000000000000000 ) ) ;
#54086=DIRECTION ( 'NONE',  ( -0.000000000000000000, 1.000000000000000000, -0.000000000000000000 ) ) ;
#54087=CONICAL_SURFACE ( 'NONE', #20649, 0.1000000000000002554, 0.003490658503988666988 ) ;
#54088=EDGE_CURVE ( 'NONE', #41131, #53209, #115456, .T. ) ;
#54089=DIRECTION ( 'NONE',  ( 0.000000000000000000, 0.000000000000000000, 1.000000000000000000 ) ) ;
#54090=FACE_OUTER_BOUND ( 'NONE', #42225, .T. ) ;
#54091=DIRECTION ( 'NONE',  ( 0.000000000000000000, 1.000000000000000000, 0.000000000000000000 ) ) ;
#54092=AXIS2_PLACEMENT_3D ( 'NONE', #12252, #56532, #111761 ) ;
#54093=DIRECTION ( 'NONE',  ( 0.000000000000000000, -0.9999939076577903929, 0.003490651415223739937 ) ) ;
#54094=ORIENTED_EDGE ( 'NONE', *, *, #44980, .T. ) ;
#54096=ORIENTED_EDGE ( 'NONE', *, *, #69373, .F. ) ;
#54097=EDGE_LOOP ( 'NONE', ( #20733, #70885 ) ) ;
#54098=ORIENTED_EDGE ( 'NONE', *, *, #14945, .F. ) ;
#54099=CONICAL_SURFACE ( 'NONE', #106333, 0.09999999999999982514, 0.003490658503988666988 ) ;
#54100=DIRECTION ( 'NONE',  ( 0.000000000000000000, 0.000000000000000000, 1.000000000000000000 ) ) ;
#54102=VERTEX_POINT ( 'NONE', #91702 ) ;
#54103=ADVANCED_FACE ( 'NONE', ( #60329 ), #23839, .T. ) ;
#54104=FACE_BOUND ( 'NONE', #87903, .T. ) ;
#54105=DIRECTION ( 'NONE',  ( -0.000000000000000000, 1.000000000000000000, -0.000000000000000000 ) ) ;
#54106=VECTOR ( 'NONE', #47584, 1000.000000000000000 ) ;
#54107=ORIENTED_EDGE ( 'NONE', *, *, #105898, .T. ) ;
#54108=CARTESIAN_POINT ( 'NONE',  ( -14.59999999999998366, 2.500000000000000000, -0.7928203230275520097 ) ) ;
#54109=EDGE_CURVE ( 'NONE', #42733, #40379, #13052, .T. ) ;
#54110=PLANE ( 'NONE',  #113847 ) ;
#54112=ORIENTED_EDGE ( 'NONE', *, *, #48385, .F. ) ;
#54113=AXIS2_PLACEMENT_3D ( 'NONE', #9413, #70267, #40166 ) ;
#54114=CARTESIAN_POINT ( 'NONE',  ( -1.900000000000034994, 12.50000000000000000, -4.676537180435978769 ) ) ;
#54115=CIRCLE ( 'NONE', #24874, 0.09999999999999982514 ) ;
#54116=ORIENTED_EDGE ( 'NONE', *, *, #93777, .F. ) ;
#54117=EDGE_LOOP ( 'NONE', ( #101544, #57883, #20359, #87730 ) ) ;
#54118=EDGE_LOOP ( 'NONE', ( #20815, #94082, #70984, #116525 ) ) ;
#54119=DIRECTION ( 'NONE',  ( 0.000000000000000000, 0.000000000000000000, -1.000000000000000000 ) ) ;
#54120=DIRECTION ( 'NONE',  ( 0.000000000000000000, 0.000000000000000000, 1.000000000000000000 ) ) ;
#54121=DIRECTION ( 'NONE',  ( -0.000000000000000000, 1.000000000000000000, -0.000000000000000000 ) ) ;
#54122=AXIS2_PLACEMENT_3D ( 'NONE', #121418, #21962, #59963 ) ;
#54123=EDGE_LOOP ( 'NONE', ( #54005, #91420, #84234, #63073 ) ) ;
#54124=LINE ( 'NONE', #94048, #5723 ) ;
#54125=FACE_OUTER_BOUND ( 'NONE', #60939, .T. ) ;
#54126=EDGE_CURVE ( 'NONE', #13704, #60192, #23537, .T. ) ;
#54127=VECTOR ( 'NONE', #65937, 1000.000000000000000 ) ;
#54128=DIRECTION ( 'NONE',  ( 0.000000000000000000, 0.000000000000000000, 1.000000000000000000 ) ) ;
#54129=CIRCLE ( 'NONE', #106355, 0.06509327318403745899 ) ;
#54131=ORIENTED_EDGE ( 'NONE', *, *, #3021, .F. ) ;
#54132=CIRCLE ( 'NONE', #97948, 0.1000000000000002554 ) ;
#54133=PLANE ( 'NONE',  #47440 ) ;
#54134=ORIENTED_EDGE ( 'NONE', *, *, #18822, .T. ) ;
#54135=LINE ( 'NONE', #75065, #54658 ) ;
#54136=ADVANCED_FACE ( 'NONE', ( #110056 ), #10542, .T. ) ;
#54137=AXIS2_PLACEMENT_3D ( 'NONE', #84273, #5702, #113091 ) ;
#54138=AXIS2_PLACEMENT_3D ( 'NONE', #83532, #13476, #82240 ) ;
#54139=ORIENTED_EDGE ( 'NONE', *, *, #18414, .F. ) ;
#54140=VERTEX_POINT ( 'NONE', #82538 ) ;
#54143=EDGE_CURVE ( 'NONE', #118512, #116743, #27739, .T. ) ;
#54144=PLANE ( 'NONE',  #11177 ) ;
#54145=CARTESIAN_POINT ( 'NONE',  ( 6.049999999999932321, 2.500000000000000000, -1.918653347947326004 ) ) ;
#54146=ADVANCED_FACE ( 'NONE', ( #30223 ), #50483, .T. ) ;
#54147=EDGE_CURVE ( 'NONE', #66596, #120245, #638, .T. ) ;
#54148=CARTESIAN_POINT ( 'NONE',  ( 8.549999999999924327, 12.50000000000000000, 1.818653347947321475 ) ) ;
#54149=EDGE_CURVE ( 'NONE', #6351, #5094, #67421, .T. ) ;
#54150=VERTEX_POINT ( 'NONE', #125650 ) ;
#54151=VERTEX_POINT ( 'NONE', #124390 ) ;
#54152=DIRECTION ( 'NONE',  ( 0.000000000000000000, 0.000000000000000000, 1.000000000000000000 ) ) ;
#54153=CARTESIAN_POINT ( 'NONE',  ( 4.349999999999937472, 12.50000000000000000, 6.841600689897072485 ) ) ;
#54154=ADVANCED_FACE ( 'NONE', ( #34737 ), #92998, .T. ) ;
#54155=DIRECTION ( 'NONE',  ( -0.000000000000000000, -1.000000000000000000, -0.000000000000000000 ) ) ;
#54156=AXIS2_PLACEMENT_3D ( 'NONE', #68586, #56184, #55558 ) ;
#54157=ORIENTED_EDGE ( 'NONE', *, *, #79852, .T. ) ;
#54158=ORIENTED_EDGE ( 'NONE', *, *, #119319, .T. ) ;
#54159=ADVANCED_FACE ( 'NONE', ( #115842 ), #48688, .T. ) ;
#54160=CARTESIAN_POINT ( 'NONE',  ( -12.04999999999999538, 12.50000000000000000, 6.495190528383297135 ) ) ;
#54162=CARTESIAN_POINT ( 'NONE',  ( -6.050000000000017586, 12.50000000000000000, 6.148780366869520009 ) ) ;
#54163=ADVANCED_FACE ( 'NONE', ( #104721 ), #121825, .T. ) ;
#54164=CONICAL_SURFACE ( 'NONE', #87588, 0.1000000000000002554, 0.003490658503988666988 ) ;
#54165=ADVANCED_FACE ( 'NONE', ( #85733 ), #42433, .T. ) ;
#54166=CIRCLE ( 'NONE', #129493, 0.1000000000000000472 ) ;
#54167=CARTESIAN_POINT ( 'NONE',  ( -1.450000000000035927, 12.50000000000000000, -1.818653347947326138 ) ) ;
#54168=EDGE_LOOP ( 'NONE', ( #75329, #16009, #84306, #60937 ) ) ;
#54169=CARTESIAN_POINT ( 'NONE',  ( 2.099999999999947686, 2.500000000000000000, 5.122947341949749323 ) ) ;
#54170=DIRECTION ( 'NONE',  ( 0.000000000000000000, 1.000000000000000000, 0.000000000000000000 ) ) ;
#54171=DIRECTION ( 'NONE',  ( 0.000000000000000000, 0.000000000000000000, -1.000000000000000000 ) ) ;
#54173=EDGE_CURVE ( 'NONE', #114385, #80836, #21489, .T. ) ;
#54174=AXIS2_PLACEMENT_3D ( 'NONE', #125974, #36345, #6825 ) ;
#54175=ORIENTED_EDGE ( 'NONE', *, *, #54861, .T. ) ;
#54176=AXIS2_PLACEMENT_3D ( 'NONE', #50303, #21482, #71887 ) ;
#54177=CONICAL_SURFACE ( 'NONE', #31201, 0.09999999999999982514, 0.003490658503988666988 ) ;
#54178=DIRECTION ( 'NONE',  ( 0.000000000000000000, -0.9999939076577903929, 0.003490651415223739937 ) ) ;
#54179=CARTESIAN_POINT ( 'NONE',  ( 76.40063402951030014, -3.742348971408897107, 5.987205606699626870 ) ) ;
#54180=VERTEX_POINT ( 'NONE', #125022 ) ;
#54181=ORIENTED_EDGE ( 'NONE', *, *, #116646, .T. ) ;
#54183=CARTESIAN_POINT ( 'NONE',  ( -10.40000000000000213, 12.50000000000000000, -5.088040615133786915 ) ) ;
#54184=DIRECTION ( 'NONE',  ( -0.000000000000000000, -1.000000000000000000, -0.000000000000000000 ) ) ;
#54185=AXIS2_PLACEMENT_3D ( 'NONE', #80816, #2224, #42171 ) ;
#54186=CARTESIAN_POINT ( 'NONE',  ( -12.89999999999999147, 2.500000000000000000, 4.330127018922196314 ) ) ;
#54187=CARTESIAN_POINT ( 'NONE',  ( -3.750000000000027978, 2.500000000000000000, 7.188010851410848723 ) ) ;
#54188=CIRCLE ( 'NONE', #125195, 0.06509327318403745899 ) ;
#54189=CARTESIAN_POINT ( 'NONE',  ( 1.899999999999951283, 12.50000000000000000, -0.3464101615137782364 ) ) ;
#54190=CARTESIAN_POINT ( 'NONE',  ( 6.649999999999930189, 12.50000000000000000, -1.537336459617587581 ) ) ;
#54191=DIRECTION ( 'NONE',  ( 0.000000000000000000, 0.000000000000000000, 1.000000000000000000 ) ) ;
#54192=CARTESIAN_POINT ( 'NONE',  ( -9.150000000000009237, 12.50000000000000000, -6.430097255199259010 ) ) ;
#54193=PLANE ( 'NONE',  #119401 ) ;
#54194=CARTESIAN_POINT ( 'NONE',  ( -6.050000000000017586, 2.500000000000000000, 6.148780366869520009 ) ) ;
#54195=ORIENTED_EDGE ( 'NONE', *, *, #77174, .T. ) ;
#54196=VERTEX_POINT ( 'NONE', #103458 ) ;
#54197=VERTEX_POINT ( 'NONE', #75272 ) ;
#54198=VECTOR ( 'NONE', #107587, 1000.000000000000000 ) ;
#54199=ORIENTED_EDGE ( 'NONE', *, *, #128803, .F. ) ;
#54200=FACE_OUTER_BOUND ( 'NONE', #101947, .T. ) ;
#54201=PLANE ( 'NONE',  #44229 ) ;
#54202=DIRECTION ( 'NONE',  ( -4.274815082592931898E-19, -0.9999939076577903929, -0.003490651415223739937 ) ) ;
#54203=ORIENTED_EDGE ( 'NONE', *, *, #71344, .T. ) ;
#54204=CARTESIAN_POINT ( 'NONE',  ( 3.149999999999944400, 2.500000000000000000, 1.818653347947321475 ) ) ;
#54205=ADVANCED_FACE ( 'NONE', ( #113267 ), #35366, .T. ) ;
#54206=EDGE_CURVE ( 'NONE', #79729, #22266, #13146, .T. ) ;
#54207=CARTESIAN_POINT ( 'NONE',  ( -8.750000000000007105, 12.50000000000000000, 7.188010851410848723 ) ) ;
#54208=DIRECTION ( 'NONE',  ( 0.000000000000000000, -0.9999939076577903929, 0.003490651415223739937 ) ) ;
#54209=ORIENTED_EDGE ( 'NONE', *, *, #76730, .F. ) ;
#54210=DIRECTION ( 'NONE',  ( 0.000000000000000000, -0.000000000000000000, 1.000000000000000000 ) ) ;
#54211=AXIS2_PLACEMENT_3D ( 'NONE', #120651, #59166, #79449 ) ;
#54212=CARTESIAN_POINT ( 'NONE',  ( -10.60000000000000320, 2.500000000000000000, -4.676537180435973440 ) ) ;
#54213=ORIENTED_EDGE ( 'NONE', *, *, #75302, .T. ) ;
#54214=ADVANCED_FACE ( 'NONE', ( #54990 ), #75854, .T. ) ;
#54216=EDGE_LOOP ( 'NONE', ( #83582, #54749, #78802, #103317 ) ) ;
#54217=ORIENTED_EDGE ( 'NONE', *, *, #28056, .T. ) ;
#54218=DIRECTION ( 'NONE',  ( -4.274815082592931898E-19, -0.9999939076577903929, -0.003490651415223739937 ) ) ;
#54219=AXIS2_PLACEMENT_3D ( 'NONE', #50592, #59813, #21135 ) ;
#54220=LINE ( 'NONE', #113787, #32109 ) ;
#54221=PLANE ( 'NONE',  #50427 ) ;
#54222=CARTESIAN_POINT ( 'NONE',  ( 0.6499999999999561684, 2.500000000000000000, -2.411473670974877859 ) ) ;
#54223=EDGE_LOOP ( 'NONE', ( #24542, #37410, #55007, #108343 ) ) ;
#54224=AXIS2_PLACEMENT_3D ( 'NONE', #29261, #108439, #116962 ) ;
#54225=AXIS2_PLACEMENT_3D ( 'NONE', #84175, #94006, #14767 ) ;
#54226=DIRECTION ( 'NONE',  ( 0.000000000000000000, 0.000000000000000000, 1.000000000000000000 ) ) ;
#54227=VERTEX_POINT ( 'NONE', #123098 ) ;
#54228=DIRECTION ( 'NONE',  ( -0.000000000000000000, -1.000000000000000000, -0.000000000000000000 ) ) ;
#54229=DIRECTION ( 'NONE',  ( -4.274815082592931898E-19, -0.9999939076577903929, -0.003490651415223739937 ) ) ;
#54230=CARTESIAN_POINT ( 'NONE',  ( -6.650000000000018119, 2.500000000000000000, -2.165063509461101710 ) ) ;
#54231=CARTESIAN_POINT ( 'NONE',  ( -7.300000000000018474, 2.500000000000000000, 0.4464101615137735513 ) ) ;
#54232=ORIENTED_EDGE ( 'NONE', *, *, #67387, .F. ) ;
#54233=AXIS2_PLACEMENT_3D ( 'NONE', #26655, #116942, #48223 ) ;
#54234=CIRCLE ( 'NONE', #12451, 0.1000000000000000472 ) ;
#54235=ORIENTED_EDGE ( 'NONE', *, *, #18333, .F. ) ;
#54236=VERTEX_POINT ( 'NONE', #93636 ) ;
#54237=DIRECTION ( 'NONE',  ( -0.000000000000000000, 1.000000000000000000, -0.000000000000000000 ) ) ;
#54238=CARTESIAN_POINT ( 'NONE',  ( -4.400000000000025224, 12.50000000000000000, 4.048810130592458201 ) ) ;
#54239=CARTESIAN_POINT ( 'NONE',  ( -11.64999999999999680, 2.500000000000000000, 2.265063509461097357 ) ) ;
#54240=FACE_BOUND ( 'NONE', #128339, .T. ) ;
#54241=DIRECTION ( 'NONE',  ( 0.000000000000000000, 1.000000000000000000, 0.000000000000000000 ) ) ;
#54242=FACE_OUTER_BOUND ( 'NONE', #107379, .T. ) ;
#54243=DIRECTION ( 'NONE',  ( -0.000000000000000000, 1.000000000000000000, -0.000000000000000000 ) ) ;
#54244=EDGE_CURVE ( 'NONE', #66584, #79607, #5874, .T. ) ;
#54245=CIRCLE ( 'NONE', #64698, 0.1000000000000002554 ) ;
#54247=CARTESIAN_POINT ( 'NONE',  ( 2.949999999999946887, 2.500000000000000000, -6.495190528383302464 ) ) ;
#54248=DIRECTION ( 'NONE',  ( 0.000000000000000000, 0.000000000000000000, 1.000000000000000000 ) ) ;
#54249=ORIENTED_EDGE ( 'NONE', *, *, #98185, .T. ) ;
#54250=AXIS2_PLACEMENT_3D ( 'NONE', #112473, #22813, #70605 ) ;
#54251=CARTESIAN_POINT ( 'NONE',  ( -8.350000000000013856, 2.500000000000000000, -6.495190528383297135 ) ) ;
#54252=ORIENTED_EDGE ( 'NONE', *, *, #4601, .F. ) ;
#54253=ORIENTED_EDGE ( 'NONE', *, *, #76470, .F. ) ;
#54254=VERTEX_POINT ( 'NONE', #55641 ) ;
#54255=VERTEX_POINT ( 'NONE', #14412 ) ;
#54256=EDGE_CURVE ( 'NONE', #65457, #34347, #29901, .T. ) ;
#54257=DIRECTION ( 'NONE',  ( 0.000000000000000000, 1.000000000000000000, 0.000000000000000000 ) ) ;
#54258=FACE_BOUND ( 'NONE', #55343, .T. ) ;
#54259=CARTESIAN_POINT ( 'NONE',  ( 2.049999999999950084, 12.50000000000000000, 2.165063509461097713 ) ) ;
#54260=CIRCLE ( 'NONE', #58482, 0.06509327318403745899 ) ;
#54261=VECTOR ( 'NONE', #27271, 1000.000000000000000 ) ;
#54262=CIRCLE ( 'NONE', #110397, 0.09999999999999982514 ) ;
#54263=VERTEX_POINT ( 'NONE', #85094 ) ;
#54264=DIRECTION ( 'NONE',  ( -4.274815082592931898E-19, -0.9999939076577903929, -0.003490651415223739937 ) ) ;
#54265=EDGE_CURVE ( 'NONE', #7939, #107780, #38229, .T. ) ;
#54266=CARTESIAN_POINT ( 'NONE',  ( -5.600000000000020073, 12.50000000000000000, 4.741630453620009789 ) ) ;
#54267=CIRCLE ( 'NONE', #52218, 0.1000000000000002554 ) ;
#54268=ORIENTED_EDGE ( 'NONE', *, *, #68158, .F. ) ;
#54269=CARTESIAN_POINT ( 'NONE',  ( -12.09999999999999609, 12.50000000000000000, 4.330127018922196314 ) ) ;
#54270=CARTESIAN_POINT ( 'NONE',  ( -14.59999999999998366, 2.500000000000000000, -1.084202172485504434E-16 ) ) ;
#54271=AXIS2_PLACEMENT_3D ( 'NONE', #2844, #4115, #102971 ) ;
#54272=AXIS2_PLACEMENT_3D ( 'NONE', #44083, #44743, #34287 ) ;
#54273=ORIENTED_EDGE ( 'NONE', *, *, #96260, .T. ) ;
#54274=DIRECTION ( 'NONE',  ( -0.000000000000000000, -1.000000000000000000, -0.000000000000000000 ) ) ;
#54275=CARTESIAN_POINT ( 'NONE',  ( 4.999999999999936939, 12.50000000000000000, -0.6277270498435166823 ) ) ;
#54276=VERTEX_POINT ( 'NONE', #95571 ) ;
#54277=DIRECTION ( 'NONE',  ( -0.000000000000000000, 1.000000000000000000, -0.000000000000000000 ) ) ;
#54279=FACE_OUTER_BOUND ( 'NONE', #307, .T. ) ;
#54280=AXIS2_PLACEMENT_3D ( 'NONE', #91169, #98392, #69588 ) ;
#54281=ORIENTED_EDGE ( 'NONE', *, *, #17806, .F. ) ;
#54282=EDGE_LOOP ( 'NONE', ( #42073, #98884, #58366, #65785 ) ) ;
#54283=CARTESIAN_POINT ( 'NONE',  ( 9.399999999999915090, 2.500000000000000000, -4.576537180435977348 ) ) ;
#54284=ORIENTED_EDGE ( 'NONE', *, *, #79864, .T. ) ;
#54285=CARTESIAN_POINT ( 'NONE',  ( -8.350000000000012079, 12.50000000000000000, -2.857883832488653741 ) ) ;
#54286=DIRECTION ( 'NONE',  ( 0.000000000000000000, 0.000000000000000000, -1.000000000000000000 ) ) ;
#54287=EDGE_CURVE ( 'NONE', #16543, #125159, #13766, .T. ) ;
#54288=ORIENTED_EDGE ( 'NONE', *, *, #84105, .F. ) ;
#54289=DIRECTION ( 'NONE',  ( 0.000000000000000000, 0.000000000000000000, 1.000000000000000000 ) ) ;
#54290=CARTESIAN_POINT ( 'NONE',  ( -7.100000000000018296, 12.50000000000000000, -4.395220292106239768 ) ) ;
#54291=DIRECTION ( 'NONE',  ( 0.000000000000000000, 0.000000000000000000, 1.000000000000000000 ) ) ;
#54292=PLANE ( 'NONE',  #88340 ) ;
#54293=EDGE_CURVE ( 'NONE', #67411, #26300, #17350, .T. ) ;
#54294=CARTESIAN_POINT ( 'NONE',  ( 9.999999999999948486, 2.500000000000000000, 4.330127018922196314 ) ) ;
#54295=EDGE_CURVE ( 'NONE', #101138, #69331, #24249, .T. ) ;
#54296=ORIENTED_EDGE ( 'NONE', *, *, #58968, .F. ) ;
#54297=ORIENTED_EDGE ( 'NONE', *, *, #75560, .T. ) ;
#54298=DIRECTION ( 'NONE',  ( 0.000000000000000000, 0.000000000000000000, 1.000000000000000000 ) ) ;
#54299=LINE ( 'NONE', #11795, #1263 ) ;
#54300=EDGE_CURVE ( 'NONE', #8031, #63281, #11007, .T. ) ;
#54301=DIRECTION ( 'NONE',  ( 0.000000000000000000, -0.9999939076577903929, 0.003490651415223739937 ) ) ;
#54302=VERTEX_POINT ( 'NONE', #68033 ) ;
#54303=VERTEX_POINT ( 'NONE', #26186 ) ;
#54304=EDGE_CURVE ( 'NONE', #83081, #39693, #37936, .T. ) ;
#54305=ORIENTED_EDGE ( 'NONE', *, *, #19381, .T. ) ;
#54306=CIRCLE ( 'NONE', #39753, 0.06509327318403745899 ) ;
#54307=EDGE_CURVE ( 'NONE', #50596, #5370, #128102, .T. ) ;
#54308=DIRECTION ( 'NONE',  ( 0.000000000000000000, 0.000000000000000000, 1.000000000000000000 ) ) ;
#54309=DIRECTION ( 'NONE',  ( 0.000000000000000000, 0.000000000000000000, 1.000000000000000000 ) ) ;
#54310=LINE ( 'NONE', #4531, #53930 ) ;
#54312=CIRCLE ( 'NONE', #27126, 0.06509327318403745899 ) ;
#54313=AXIS2_PLACEMENT_3D ( 'NONE', #96562, #77571, #18012 ) ;
#54314=EDGE_CURVE ( 'NONE', #103678, #91712, #79169, .T. ) ;
#54315=DIRECTION ( 'NONE',  ( -4.274815082592931898E-19, -0.9999939076577903929, -0.003490651415223739937 ) ) ;
#54317=CARTESIAN_POINT ( 'NONE',  ( 11.84999999999990727, 12.50000000000000000, -1.753560074763288679 ) ) ;
#54318=DIRECTION ( 'NONE',  ( 0.000000000000000000, 0.000000000000000000, 1.000000000000000000 ) ) ;
#54319=DIRECTION ( 'NONE',  ( 0.000000000000000000, 1.000000000000000000, 0.000000000000000000 ) ) ;
#54320=AXIS2_PLACEMENT_3D ( 'NONE', #56519, #6745, #59115 ) ;
#54321=LINE ( 'NONE', #35334, #102103 ) ;
#54322=ADVANCED_FACE ( 'NONE', ( #18922 ), #96777, .T. ) ;
#54324=VERTEX_POINT ( 'NONE', #96843 ) ;
#54325=DIRECTION ( 'NONE',  ( -0.000000000000000000, 1.000000000000000000, -0.000000000000000000 ) ) ;
#54326=VERTEX_POINT ( 'NONE', #128923 ) ;
#54327=ORIENTED_EDGE ( 'NONE', *, *, #55703, .T. ) ;
#54328=CARTESIAN_POINT ( 'NONE',  ( -7.050000000000013145, 2.500000000000000000, 2.165063509461097713 ) ) ;
#54329=CARTESIAN_POINT ( 'NONE',  ( 10.84999999999991260, 12.50000000000000000, -1.537336459617587581 ) ) ;
#54330=FACE_OUTER_BOUND ( 'NONE', #121816, .T. ) ;
#54331=DIRECTION ( 'NONE',  ( 0.000000000000000000, 0.000000000000000000, 1.000000000000000000 ) ) ;
#54332=DIRECTION ( 'NONE',  ( 0.000000000000000000, 0.000000000000000000, 1.000000000000000000 ) ) ;
#54333=CARTESIAN_POINT ( 'NONE',  ( -1.250000000000037526, 2.500000000000000000, -1.572243186433550211 ) ) ;
#54334=FACE_OUTER_BOUND ( 'NONE', #120924, .T. ) ;
#54335=ORIENTED_EDGE ( 'NONE', *, *, #81891, .T. ) ;
#54337=FACE_OUTER_BOUND ( 'NONE', #18077, .T. ) ;
#54338=ORIENTED_EDGE ( 'NONE', *, *, #24370, .F. ) ;
#54339=CIRCLE ( 'NONE', #81534, 0.06509327318403745899 ) ;
#54340=ORIENTED_EDGE ( 'NONE', *, *, #52984, .F. ) ;
#54341=EDGE_LOOP ( 'NONE', ( #89546, #110453, #36001, #85504 ) ) ;
#54342=ORIENTED_EDGE ( 'NONE', *, *, #17973, .F. ) ;
#54343=DIRECTION ( 'NONE',  ( 0.000000000000000000, 0.000000000000000000, 1.000000000000000000 ) ) ;
#54344=CARTESIAN_POINT ( 'NONE',  ( 12.29999999999990479, 2.500000000000000000, -3.983716857408426293 ) ) ;
#54345=CIRCLE ( 'NONE', #14610, 0.06509327318403745899 ) ;
#54346=DIRECTION ( 'NONE',  ( 0.000000000000000000, 1.000000000000000000, 0.000000000000000000 ) ) ;
#54347=EDGE_CURVE ( 'NONE', #43713, #48486, #31970, .T. ) ;
#54348=DIRECTION ( 'NONE',  ( -0.000000000000000000, 1.000000000000000000, -0.000000000000000000 ) ) ;
#54349=CARTESIAN_POINT ( 'NONE',  ( 5.649999999999936406, 2.500000000000000000, -6.841600689897077814 ) ) ;
#54350=ORIENTED_EDGE ( 'NONE', *, *, #106721, .F. ) ;
#54351=FACE_OUTER_BOUND ( 'NONE', #5140, .T. ) ;
#54352=LINE ( 'NONE', #124395, #107986 ) ;
#54353=AXIS2_PLACEMENT_3D ( 'NONE', #75981, #56330, #118325 ) ;
#54354=CARTESIAN_POINT ( 'NONE',  ( 7.899999999999924860, 2.500000000000000000, -3.737306695894649700 ) ) ;
#54355=ADVANCED_FACE ( 'NONE', ( #8453 ), #1623, .T. ) ;
#54356=CIRCLE ( 'NONE', #129606, 0.09999999999999982514 ) ;
#54357=EDGE_LOOP ( 'NONE', ( #11792, #24050 ) ) ;
#54358=CIRCLE ( 'NONE', #58579, 0.1000000000000002554 ) ;
#54359=ORIENTED_EDGE ( 'NONE', *, *, #35991, .F. ) ;
#54360=VERTEX_POINT ( 'NONE', #18287 ) ;
#54361=FACE_OUTER_BOUND ( 'NONE', #62895, .T. ) ;
#54362=CONICAL_SURFACE ( 'NONE', #94079, 0.1000000000000002554, 0.003490658503988666988 ) ;
#54363=CIRCLE ( 'NONE', #127529, 0.06509327318403745899 ) ;
#54364=CARTESIAN_POINT ( 'NONE',  ( -1.900000000000035438, 2.500000000000000000, 3.983716857408420076 ) ) ;
#54365=CARTESIAN_POINT ( 'NONE',  ( -0.8000000000000315747, 12.50000000000000000, 0.000000000000000000 ) ) ;
#54366=CIRCLE ( 'NONE', #127535, 0.1000000000000000472 ) ;
#54367=ORIENTED_EDGE ( 'NONE', *, *, #43403, .T. ) ;
#54368=DIRECTION ( 'NONE',  ( -0.000000000000000000, -1.000000000000000000, -0.000000000000000000 ) ) ;
#54369=CARTESIAN_POINT ( 'NONE',  ( -4.600000000000024514, 2.500000000000000000, -0.5928203230275542746 ) ) ;
#54370=CARTESIAN_POINT ( 'NONE',  ( 9.549999999999915445, 2.500000000000000000, -2.065063509461102065 ) ) ;
#54371=DIRECTION ( 'NONE',  ( -0.000000000000000000, 1.000000000000000000, -0.000000000000000000 ) ) ;
#54372=DIRECTION ( 'NONE',  ( 0.000000000000000000, 0.000000000000000000, 1.000000000000000000 ) ) ;
#54373=ORIENTED_EDGE ( 'NONE', *, *, #65374, .T. ) ;
#54374=ORIENTED_EDGE ( 'NONE', *, *, #35258, .T. ) ;
#54375=CARTESIAN_POINT ( 'NONE',  ( 1.049999999999954081, 2.500000000000000000, -6.148780366869526226 ) ) ;
#54376=CARTESIAN_POINT ( 'NONE',  ( 8.149999999999923972, 2.500000000000000000, -6.741600689897077281 ) ) ;
#54377=CARTESIAN_POINT ( 'NONE',  ( 12.09999999999990550, 2.500000000000000000, 3.637306695894644726 ) ) ;
#54378=LINE ( 'NONE', #74672, #125905 ) ;
#54379=DIRECTION ( 'NONE',  ( -0.000000000000000000, 1.000000000000000000, -0.000000000000000000 ) ) ;
#54380=ADVANCED_FACE ( 'NONE', ( #78529 ), #82132, .T. ) ;
#54381=EDGE_LOOP ( 'NONE', ( #57418, #5647, #79248, #113951 ) ) ;
#54382=CIRCLE ( 'NONE', #117067, 0.06509327318403745899 ) ;
#54383=VERTEX_POINT ( 'NONE', #17636 ) ;
#54384=DIRECTION ( 'NONE',  ( 0.000000000000000000, 0.000000000000000000, -1.000000000000000000 ) ) ;
#54385=AXIS2_PLACEMENT_3D ( 'NONE', #95369, #14835, #44987 ) ;
#54386=CARTESIAN_POINT ( 'NONE',  ( 6.249999999999967137, 2.500000000000000000, -2.165063509461101710 ) ) ;
#54387=DIRECTION ( 'NONE',  ( 0.000000000000000000, 0.000000000000000000, 1.000000000000000000 ) ) ;
#54388=CARTESIAN_POINT ( 'NONE',  ( 6.049999999999934097, 12.50000000000000000, -2.511473670974877948 ) ) ;
#54389=ORIENTED_EDGE ( 'NONE', *, *, #73261, .T. ) ;
#54390=EDGE_CURVE ( 'NONE', #24991, #85122, #76575, .T. ) ;
#54391=DIRECTION ( 'NONE',  ( 0.000000000000000000, -0.9999939076577903929, 0.003490651415223739937 ) ) ;
#54392=AXIS2_PLACEMENT_3D ( 'NONE', #3500, #62435, #72887 ) ;
#54393=AXIS2_PLACEMENT_3D ( 'NONE', #63755, #52005, #91920 ) ;
#54394=CARTESIAN_POINT ( 'NONE',  ( -12.69999999999999218, 2.500000000000000000, -0.3464101615137741286 ) ) ;
#54395=VERTEX_POINT ( 'NONE', #58238 ) ;
#54396=EDGE_CURVE ( 'NONE', #113036, #5090, #87028, .T. ) ;
#54397=DIRECTION ( 'NONE',  ( 0.000000000000000000, 0.000000000000000000, 1.000000000000000000 ) ) ;
#54398=EDGE_CURVE ( 'NONE', #40560, #72456, #98841, .T. ) ;
#54399=ORIENTED_EDGE ( 'NONE', *, *, #52279, .T. ) ;
#54400=DIRECTION ( 'NONE',  ( 0.000000000000000000, -0.000000000000000000, 1.000000000000000000 ) ) ;
#54401=AXIS2_PLACEMENT_3D ( 'NONE', #62892, #103462, #46295 ) ;
#54402=EDGE_LOOP ( 'NONE', ( #5421, #5056, #40346, #41214 ) ) ;
#54403=DIRECTION ( 'NONE',  ( 0.000000000000000000, -0.9999939076577903929, 0.003490651415223739937 ) ) ;
#54404=DIRECTION ( 'NONE',  ( -0.000000000000000000, 1.000000000000000000, -0.000000000000000000 ) ) ;
#54405=ADVANCED_FACE ( 'NONE', ( #118422 ), #63351, .T. ) ;
#54406=ORIENTED_EDGE ( 'NONE', *, *, #59997, .F. ) ;
#54407=VERTEX_POINT ( 'NONE', #107316 ) ;
#54410=DIRECTION ( 'NONE',  ( 0.000000000000000000, 1.000000000000000000, 0.000000000000000000 ) ) ;
#54411=DIRECTION ( 'NONE',  ( -0.000000000000000000, 1.000000000000000000, -0.000000000000000000 ) ) ;
#54412=CARTESIAN_POINT ( 'NONE',  ( 2.099999999999950351, 12.50000000000000000, -4.957854068765716882 ) ) ;
#54413=DIRECTION ( 'NONE',  ( -0.000000000000000000, 1.000000000000000000, -0.000000000000000000 ) ) ;
#54415=DIRECTION ( 'NONE',  ( 0.000000000000000000, 1.000000000000000000, 0.000000000000000000 ) ) ;
#54416=AXIS2_PLACEMENT_3D ( 'NONE', #102129, #29526, #60297 ) ;
#54417=VECTOR ( 'NONE', #122910, 1000.000000000000000 ) ;
#54418=ORIENTED_EDGE ( 'NONE', *, *, #1085, .T. ) ;
#54419=ORIENTED_EDGE ( 'NONE', *, *, #5688, .T. ) ;
#54420=CARTESIAN_POINT ( 'NONE',  ( 4.799999999999937650, 2.500000000000000000, -3.883716857408426648 ) ) ;
#54421=CARTESIAN_POINT ( 'NONE',  ( -5.000000000000023093, 12.50000000000000000, 5.088040615133786027 ) ) ;
#54422=DIRECTION ( 'NONE',  ( 0.000000000000000000, 0.000000000000000000, 1.000000000000000000 ) ) ;
#54423=FACE_OUTER_BOUND ( 'NONE', #89426, .T. ) ;
#54424=ORIENTED_EDGE ( 'NONE', *, *, #46913, .T. ) ;
#54425=VERTEX_POINT ( 'NONE', #51634 ) ;
#54426=DIRECTION ( 'NONE',  ( 0.000000000000000000, -0.9999939076577903929, 0.003490651415223739937 ) ) ;
#54427=ORIENTED_EDGE ( 'NONE', *, *, #50184, .F. ) ;
#54428=CARTESIAN_POINT ( 'NONE',  ( 11.24999999999990763, 2.500000000000000000, 1.472243186433545459 ) ) ;
#54429=DIRECTION ( 'NONE',  ( -4.274815082592931898E-19, -0.9999939076577903929, -0.003490651415223739937 ) ) ;
#54430=AXIS2_PLACEMENT_3D ( 'NONE', #113135, #35239, #4439 ) ;
#54431=EDGE_LOOP ( 'NONE', ( #57818, #34952, #39153, #121763 ) ) ;
#54432=DIRECTION ( 'NONE',  ( 0.000000000000000000, 1.000000000000000000, 0.000000000000000000 ) ) ;
#54433=CARTESIAN_POINT ( 'NONE',  ( 10.84999999999991260, 2.500000000000000000, 7.088010851410848190 ) ) ;
#54434=EDGE_CURVE ( 'NONE', #124886, #90021, #119778, .T. ) ;
#54435=DIRECTION ( 'NONE',  ( 0.000000000000000000, 0.000000000000000000, 1.000000000000000000 ) ) ;
#54436=FACE_OUTER_BOUND ( 'NONE', #82174, .T. ) ;
#54437=DIRECTION ( 'NONE',  ( 0.000000000000000000, 0.000000000000000000, -1.000000000000000000 ) ) ;
#54438=CARTESIAN_POINT ( 'NONE',  ( 10.19999999999991225, 2.500000000000000000, 3.983716857408420076 ) ) ;
#54439=CARTESIAN_POINT ( 'NONE',  ( -11.25000000000000000, 2.500000000000000000, 7.288010851410849256 ) ) ;
#54440=CARTESIAN_POINT ( 'NONE',  ( -4.999999999999990230, 12.50000000000000000, -4.395220292106239768 ) ) ;
#54441=DIRECTION ( 'NONE',  ( 0.000000000000000000, 1.000000000000000000, 0.000000000000000000 ) ) ;
#54442=EDGE_CURVE ( 'NONE', #114390, #87221, #91549, .T. ) ;
#54443=AXIS2_PLACEMENT_3D ( 'NONE', #56919, #115187, #116501 ) ;
#54444=ORIENTED_EDGE ( 'NONE', *, *, #109126, .T. ) ;
#54445=ORIENTED_EDGE ( 'NONE', *, *, #12303, .T. ) ;
#54446=CIRCLE ( 'NONE', #58666, 0.06509327318403745899 ) ;
#54447=VERTEX_POINT ( 'NONE', #21521 ) ;
#54448=DIRECTION ( 'NONE',  ( 0.000000000000000000, 0.000000000000000000, -1.000000000000000000 ) ) ;
#54449=ORIENTED_EDGE ( 'NONE', *, *, #77914, .F. ) ;
#54450=DIRECTION ( 'NONE',  ( -4.274815082592931898E-19, -0.9999939076577903929, -0.003490651415223739937 ) ) ;
#54451=ADVANCED_FACE ( 'NONE', ( #11036 ), #34107, .T. ) ;
#54452=ORIENTED_EDGE ( 'NONE', *, *, #34732, .F. ) ;
#54453=VERTEX_POINT ( 'NONE', #109908 ) ;
#54454=ORIENTED_EDGE ( 'NONE', *, *, #63725, .F. ) ;
#54455=ADVANCED_FACE ( 'NONE', ( #89615 ), #50830, .T. ) ;
#54456=FACE_OUTER_BOUND ( 'NONE', #61540, .T. ) ;
#54457=CIRCLE ( 'NONE', #96306, 0.1000000000000002554 ) ;
#54458=ADVANCED_FACE ( 'NONE', ( #1866 ), #40476, .T. ) ;
#54459=CARTESIAN_POINT ( 'NONE',  ( -11.05000000000000071, 2.500000000000000000, -6.841600689897075149 ) ) ;
#54461=EDGE_CURVE ( 'NONE', #26094, #127992, #41824, .T. ) ;
#54463=LINE ( 'NONE', #2142, #87694 ) ;
#54464=FACE_OUTER_BOUND ( 'NONE', #47873, .T. ) ;
#54465=EDGE_LOOP ( 'NONE', ( #49926, #26009, #38463, #6139 ) ) ;
#54466=CARTESIAN_POINT ( 'NONE',  ( 11.04999999999990834, 2.500000000000000000, -6.741600689897077281 ) ) ;
#54467=ADVANCED_FACE ( 'NONE', ( #100082 ), #124071, .T. ) ;
#54469=EDGE_CURVE ( 'NONE', #18441, #9509, #86407, .T. ) ;
#54470=ORIENTED_EDGE ( 'NONE', *, *, #74885, .T. ) ;
#54471=ORIENTED_EDGE ( 'NONE', *, *, #78837, .F. ) ;
#54472=DIRECTION ( 'NONE',  ( 0.000000000000000000, 0.000000000000000000, 1.000000000000000000 ) ) ;
#54473=ORIENTED_EDGE ( 'NONE', *, *, #117889, .F. ) ;
#54474=VERTEX_POINT ( 'NONE', #110537 ) ;
#54475=EDGE_LOOP ( 'NONE', ( #88576, #50329 ) ) ;
#54477=DIRECTION ( 'NONE',  ( 0.000000000000000000, 0.000000000000000000, -1.000000000000000000 ) ) ;
#54478=DIRECTION ( 'NONE',  ( 0.000000000000000000, 0.000000000000000000, 1.000000000000000000 ) ) ;
#54479=FACE_OUTER_BOUND ( 'NONE', #36659, .T. ) ;
#54480=DIRECTION ( 'NONE',  ( 0.000000000000000000, 0.000000000000000000, 1.000000000000000000 ) ) ;
#54481=AXIS2_PLACEMENT_3D ( 'NONE', #61590, #22315, #22944 ) ;
#54482=CARTESIAN_POINT ( 'NONE',  ( -3.950000000000026379, 12.50000000000000000, 2.576566944158910744 ) ) ;
#54483=ORIENTED_EDGE ( 'NONE', *, *, #95922, .T. ) ;
#54484=AXIS2_PLACEMENT_3D ( 'NONE', #44041, #4096, #93784 ) ;
#54486=DIRECTION ( 'NONE',  ( -0.000000000000000000, -1.000000000000000000, -0.000000000000000000 ) ) ;
#54487=ORIENTED_EDGE ( 'NONE', *, *, #81459, .T. ) ;
#54488=FACE_OUTER_BOUND ( 'NONE', #21627, .T. ) ;
#54489=ORIENTED_EDGE ( 'NONE', *, *, #125271, .T. ) ;
#54490=DIRECTION ( 'NONE',  ( 0.000000000000000000, 0.000000000000000000, 1.000000000000000000 ) ) ;
#54491=VERTEX_POINT ( 'NONE', #79790 ) ;
#54492=CIRCLE ( 'NONE', #31513, 0.06509327318403745899 ) ;
#54493=ORIENTED_EDGE ( 'NONE', *, *, #4630, .T. ) ;
#54494=DIRECTION ( 'NONE',  ( -0.000000000000000000, -1.000000000000000000, -0.000000000000000000 ) ) ;
#54495=CARTESIAN_POINT ( 'NONE',  ( 3.349999999999945466, 12.50000000000000000, -2.857883832488653741 ) ) ;
#54496=CARTESIAN_POINT ( 'NONE',  ( -1.650000000000034772, 2.500000000000000000, 1.572243186433545548 ) ) ;
#54497=ORIENTED_EDGE ( 'NONE', *, *, #26729, .F. ) ;
#54498=DIRECTION ( 'NONE',  ( 0.000000000000000000, 0.000000000000000000, 1.000000000000000000 ) ) ;
#54499=VERTEX_POINT ( 'NONE', #574 ) ;
#54500=DIRECTION ( 'NONE',  ( -0.000000000000000000, -1.000000000000000000, -0.000000000000000000 ) ) ;
#54501=LINE ( 'NONE', #94422, #49450 ) ;
#54502=CARTESIAN_POINT ( 'NONE',  ( -0.8500000000000386136, 12.50000000000000000, 7.188010851410848723 ) ) ;
#54503=CARTESIAN_POINT ( 'NONE',  ( -9.999999999999969802, 12.50000000000000000, -2.276824562219559311E-15 ) ) ;
#54504=CARTESIAN_POINT ( 'NONE',  ( -9.800000000000004263, 2.500000000000000000, 3.883716857408420431 ) ) ;
#54505=EDGE_CURVE ( 'NONE', #75521, #23353, #100998, .T. ) ;
#54506=VERTEX_POINT ( 'NONE', #30064 ) ;
#54507=ORIENTED_EDGE ( 'NONE', *, *, #8294, .T. ) ;
#54508=LINE ( 'NONE', #122626, #105059 ) ;
#54509=AXIS2_PLACEMENT_3D ( 'NONE', #36808, #57067, #37453 ) ;
#54510=FACE_OUTER_BOUND ( 'NONE', #48775, .T. ) ;
#54511=AXIS2_PLACEMENT_3D ( 'NONE', #88778, #29228, #50787 ) ;
#54513=CARTESIAN_POINT ( 'NONE',  ( -0.6000000000000383915, 12.50000000000000000, -4.676537180435977881 ) ) ;
#54514=LINE ( 'NONE', #23134, #75904 ) ;
#54515=PLANE ( 'NONE',  #98302 ) ;
#54516=CARTESIAN_POINT ( 'NONE',  ( 2.049999999999950084, 12.50000000000000000, -2.099970236277064473 ) ) ;
#54517=ORIENTED_EDGE ( 'NONE', *, *, #75888, .F. ) ;
#54518=AXIS2_PLACEMENT_3D ( 'NONE', #22044, #61961, #110398 ) ;
#54519=AXIS2_PLACEMENT_3D ( 'NONE', #74777, #25030, #105526 ) ;
#54520=CARTESIAN_POINT ( 'NONE',  ( -0.4500000000000402012, 12.50000000000000000, 2.165063509461097713 ) ) ;
#54521=CARTESIAN_POINT ( 'NONE',  ( 11.24999999999994316, 2.500000000000000000, -6.495190528383302464 ) ) ;
#54522=DIRECTION ( 'NONE',  ( -0.000000000000000000, -1.000000000000000000, -0.000000000000000000 ) ) ;
#54523=VERTEX_POINT ( 'NONE', #69980 ) ;
#54524=DIRECTION ( 'NONE',  ( 0.000000000000000000, 0.000000000000000000, 1.000000000000000000 ) ) ;
#54525=CONICAL_SURFACE ( 'NONE', #10602, 0.1000000000000002554, 0.003490658503988666988 ) ;
#54526=VERTEX_POINT ( 'NONE', #60173 ) ;
#54527=CARTESIAN_POINT ( 'NONE',  ( 5.199999999999935341, 2.500000000000000000, -3.983716857408426293 ) ) ;
#54528=ORIENTED_EDGE ( 'NONE', *, *, #84427, .T. ) ;
#54529=CARTESIAN_POINT ( 'NONE',  ( -0.6500000000000394351, 2.500000000000000000, 6.841600689897072485 ) ) ;
#54530=DIRECTION ( 'NONE',  ( 0.000000000000000000, -0.9999939076577903929, 0.003490651415223739937 ) ) ;
#54531=DIRECTION ( 'NONE',  ( -0.000000000000000000, 1.000000000000000000, -0.000000000000000000 ) ) ;
#54532=ORIENTED_EDGE ( 'NONE', *, *, #64224, .F. ) ;
#54533=EDGE_CURVE ( 'NONE', #19040, #39809, #21580, .T. ) ;
#54536=CONICAL_SURFACE ( 'NONE', #60822, 0.09999999999999982514, 0.003490658503988666988 ) ;
#54537=EDGE_CURVE ( 'NONE', #4682, #44082, #84267, .T. ) ;
#54538=EDGE_CURVE ( 'NONE', #51372, #2839, #34210, .T. ) ;
#54539=ORIENTED_EDGE ( 'NONE', *, *, #44603, .T. ) ;
#54540=DIRECTION ( 'NONE',  ( -0.000000000000000000, 1.000000000000000000, -0.000000000000000000 ) ) ;
#54541=VERTEX_POINT ( 'NONE', #128026 ) ;
#54542=ORIENTED_EDGE ( 'NONE', *, *, #48116, .F. ) ;
#54543=CARTESIAN_POINT ( 'NONE',  ( -4.150000000000024336, 12.50000000000000000, 2.230156782645134950 ) ) ;
#54544=DIRECTION ( 'NONE',  ( 0.000000000000000000, 1.000000000000000000, 0.000000000000000000 ) ) ;
#54545=EDGE_CURVE ( 'NONE', #33567, #63146, #50932, .T. ) ;
#54546=EDGE_CURVE ( 'NONE', #26182, #49424, #27830, .T. ) ;
#54547=DIRECTION ( 'NONE',  ( 0.000000000000000000, 1.000000000000000000, 0.000000000000000000 ) ) ;
#54548=ADVANCED_FACE ( 'NONE', ( #27237 ), #57176, .T. ) ;
#54549=ORIENTED_EDGE ( 'NONE', *, *, #114069, .T. ) ;
#54550=EDGE_CURVE ( 'NONE', #14780, #121980, #126130, .T. ) ;
#54551=CARTESIAN_POINT ( 'NONE',  ( -6.050000000000018474, 12.50000000000000000, 2.576566944158910744 ) ) ;
#54552=CARTESIAN_POINT ( 'NONE',  ( 12.09999999999990550, 12.50000000000000000, 3.572213422710607489 ) ) ;
#54553=VERTEX_POINT ( 'NONE', #49488 ) ;
#54554=DIRECTION ( 'NONE',  ( -0.000000000000000000, -1.000000000000000000, -0.000000000000000000 ) ) ;
#54555=DIRECTION ( 'NONE',  ( 0.000000000000000000, 0.000000000000000000, 1.000000000000000000 ) ) ;
#54556=CIRCLE ( 'NONE', #58786, 0.06509327318403745899 ) ;
#54557=DIRECTION ( 'NONE',  ( 0.000000000000000000, 1.000000000000000000, 0.000000000000000000 ) ) ;
#54558=DIRECTION ( 'NONE',  ( 0.000000000000000000, 0.000000000000000000, 1.000000000000000000 ) ) ;
#54559=CARTESIAN_POINT ( 'NONE',  ( 12.09999999999990550, 2.500000000000000000, -5.122947341949753763 ) ) ;
#54560=AXIS2_PLACEMENT_3D ( 'NONE', #28918, #68172, #107465 ) ;
#54561=CIRCLE ( 'NONE', #106884, 0.06509327318403745899 ) ;
#54562=CARTESIAN_POINT ( 'NONE',  ( -11.24999999999999822, 12.50000000000000000, 1.472243186433545459 ) ) ;
#54563=LINE ( 'NONE', #75495, #31667 ) ;
#54564=CIRCLE ( 'NONE', #117250, 0.09999999999999982514 ) ;
#54565=VERTEX_POINT ( 'NONE', #126745 ) ;
#54566=ORIENTED_EDGE ( 'NONE', *, *, #62458, .F. ) ;
#54567=ORIENTED_EDGE ( 'NONE', *, *, #30718, .T. ) ;
#54568=EDGE_LOOP ( 'NONE', ( #40148, #107259 ) ) ;
#54569=DIRECTION ( 'NONE',  ( 0.000000000000000000, 0.000000000000000000, -1.000000000000000000 ) ) ;
#54570=CARTESIAN_POINT ( 'NONE',  ( 6.649999999999928413, 2.500000000000000000, 2.857883832488649301 ) ) ;
#54571=AXIS2_PLACEMENT_3D ( 'NONE', #79587, #117542, #69109 ) ;
#54572=FACE_OUTER_BOUND ( 'NONE', #116056, .T. ) ;
#54573=ORIENTED_EDGE ( 'NONE', *, *, #95252, .T. ) ;
#54574=FACE_BOUND ( 'NONE', #7502, .T. ) ;
#54575=CARTESIAN_POINT ( 'NONE',  ( -10.00000000000000533, 2.500000000000000000, -4.922947341949749145 ) ) ;
#54576=LINE ( 'NONE', #44789, #100203 ) ;
#54577=DIRECTION ( 'NONE',  ( 0.000000000000000000, -0.000000000000000000, 1.000000000000000000 ) ) ;
#54578=DIRECTION ( 'NONE',  ( -0.000000000000000000, 1.000000000000000000, -0.000000000000000000 ) ) ;
#54579=DIRECTION ( 'NONE',  ( -0.000000000000000000, 1.000000000000000000, -0.000000000000000000 ) ) ;
#54580=FACE_OUTER_BOUND ( 'NONE', #117823, .T. ) ;
#54581=PLANE ( 'NONE',  #112325 ) ;
#54582=FACE_OUTER_BOUND ( 'NONE', #13605, .T. ) ;
#54583=EDGE_CURVE ( 'NONE', #42141, #76556, #25782, .T. ) ;
#54584=DIRECTION ( 'NONE',  ( -0.000000000000000000, 1.000000000000000000, -0.000000000000000000 ) ) ;
#54585=CARTESIAN_POINT ( 'NONE',  ( 10.39999999999991154, 12.50000000000000000, 3.637306695894644726 ) ) ;
#54586=AXIS2_PLACEMENT_3D ( 'NONE', #24833, #5174, #112580 ) ;
#54587=ORIENTED_EDGE ( 'NONE', *, *, #18496, .F. ) ;
#54588=ORIENTED_EDGE ( 'NONE', *, *, #95412, .T. ) ;
#54589=VERTEX_POINT ( 'NONE', #89394 ) ;
#54590=ORIENTED_EDGE ( 'NONE', *, *, #42241, .T. ) ;
#54591=LINE ( 'NONE', #125914, #43644 ) ;
#54592=VERTEX_POINT ( 'NONE', #129342 ) ;
#54593=ADVANCED_FACE ( 'NONE', ( #106448 ), #23741, .T. ) ;
#54594=FACE_OUTER_BOUND ( 'NONE', #125065, .T. ) ;
#54595=ADVANCED_FACE ( 'NONE', ( #29203 ), #105198, .T. ) ;
#54596=EDGE_LOOP ( 'NONE', ( #60790, #117126, #66360, #16892 ) ) ;
#54597=EDGE_LOOP ( 'NONE', ( #52131, #69414, #108159, #89893 ) ) ;
#54598=EDGE_CURVE ( 'NONE', #63919, #14173, #117698, .T. ) ;
#54599=CIRCLE ( 'NONE', #94405, 0.06509327318403745899 ) ;
#54600=CARTESIAN_POINT ( 'NONE',  ( 10.63722763381580272, -2.499999999999999112, 8.014330155767860120 ) ) ;
#54601=CARTESIAN_POINT ( 'NONE',  ( 13.14999999999989733, 2.500000000000000000, -2.611473670974877592 ) ) ;
#54602=CARTESIAN_POINT ( 'NONE',  ( 9.999999999999911182, 2.500000000000000000, -3.737306695894649700 ) ) ;
#54603=EDGE_CURVE ( 'NONE', #93230, #51306, #68448, .T. ) ;
#54604=CARTESIAN_POINT ( 'NONE',  ( 11.24999999999994493, 2.500000000000000000, -2.065063509461102065 ) ) ;
#54605=EDGE_CURVE ( 'NONE', #91647, #13873, #2800, .T. ) ;
#54606=( BOUNDED_SURFACE ( )  B_SPLINE_SURFACE ( 3, 2, ( 
 ( #73603, #21286, #71681 ),
 ( #71042, #120779, #123360 ),
 ( #113537, #122719, #33693 ),
 ( #32435, #121417, #21961 ),
 ( #23887, #61880, #22606 ),
 ( #110942, #62525, #2281 ),
 ( #43531, #63804, #61222 ),
 ( #102437, #52054, #92613 ),
 ( #101149, #33069, #13394 ),
 ( #103732, #14031, #53976 ),
 ( #93908, #4211, #126591 ),
 ( #25150, #95837, #54600 ),
 ( #46739, #86654, #95193 ),
 ( #125296, #123996, #5500 ),
 ( #6775, #104363, #75532 ),
 ( #94536, #116749, #6148 ),
 ( #14674, #36926, #104990 ),
 ( #96458, #67000, #97121 ),
 ( #45464, #76847, #4858 ),
 ( #44813, #36292, #27098 ) ),
 .UNSPECIFIED., .F., .F., .F. ) 
 B_SPLINE_SURFACE_WITH_KNOTS ( ( 4, 2, 2, 2, 2, 2, 2, 2, 2, 4 ),
 ( 3, 3 ),
 ( 9.383769802862040876E-17, 0.0008832438798942619709, 0.001766487759788430050, 0.002649731639682598346, 0.003532975519576766425, 0.005299463279365103016, 0.007065951039153439174, 0.008832438798941775332, 0.01059892655873011236, 0.01413190207830678467 ),
 ( 0.000000000000000000, 1.000000000000000000 ),
 .UNSPECIFIED. ) 
 GEOMETRIC_REPRESENTATION_ITEM ( )  RATIONAL_B_SPLINE_SURFACE ( (
 ( 1.000000000000000000, 0.7071067811865477948, 1.000000000000000000),
 ( 1.000000000000000000, 0.7071067811865477948, 1.000000000000000000),
 ( 1.000000000000000000, 0.7071067811865471286, 1.000000000000000000),
 ( 1.000000000000000000, 0.7071067811865471286, 1.000000000000000000),
 ( 1.000000000000000000, 0.7071067811865477948, 1.000000000000000000),
 ( 1.000000000000000000, 0.7071067811865477948, 1.000000000000000000),
 ( 1.000000000000000000, 0.7071067811865476838, 1.000000000000000000),
 ( 1.000000000000000000, 0.7071067811865476838, 1.000000000000000000),
 ( 1.000000000000000000, 0.7071067811865472397, 1.000000000000000000),
 ( 1.000000000000000000, 0.7071067811865472397, 1.000000000000000000),
 ( 1.000000000000000000, 0.7071067811865474617, 1.000000000000000000),
 ( 1.000000000000000000, 0.7071067811865474617, 1.000000000000000000),
 ( 1.000000000000000000, 0.7071067811865474617, 1.000000000000000000),
 ( 1.000000000000000000, 0.7071067811865474617, 1.000000000000000000),
 ( 1.000000000000000000, 0.7071067811865477948, 1.000000000000000000),
 ( 1.000000000000000000, 0.7071067811865477948, 1.000000000000000000),
 ( 1.000000000000000000, 0.7071067811865473507, 1.000000000000000000),
 ( 1.000000000000000000, 0.7071067811865473507, 1.000000000000000000),
 ( 1.000000000000000000, 0.7071067811865472397, 1.000000000000000000),
 ( 1.000000000000000000, 0.7071067811865472397, 1.000000000000000000) ) ) 
 REPRESENTATION_ITEM ( '' )  SURFACE ( )  );
#54607=ORIENTED_EDGE ( 'NONE', *, *, #83650, .F. ) ;
#54608=CONICAL_SURFACE ( 'NONE', #71329, 0.1000000000000002554, 0.003490658503988666988 ) ;
#54609=EDGE_CURVE ( 'NONE', #1900, #126243, #107344, .T. ) ;
#54610=AXIS2_PLACEMENT_3D ( 'NONE', #7144, #47105, #54968 ) ;
#54611=ADVANCED_FACE ( 'NONE', ( #29830 ), #61299, .T. ) ;
#54612=ORIENTED_EDGE ( 'NONE', *, *, #80188, .T. ) ;
#54613=EDGE_CURVE ( 'NONE', #103318, #126889, #39036, .T. ) ;
#54614=VERTEX_POINT ( 'NONE', #76991 ) ;
#54615=CARTESIAN_POINT ( 'NONE',  ( 1.849999999999949685, 12.50000000000000000, -2.511473670974877948 ) ) ;
#54616=ORIENTED_EDGE ( 'NONE', *, *, #62602, .T. ) ;
#54618=ORIENTED_EDGE ( 'NONE', *, *, #54613, .T. ) ;
#54619=ORIENTED_EDGE ( 'NONE', *, *, #22245, .F. ) ;
#54620=ADVANCED_FACE ( 'NONE', ( #57351 ), #97273, .T. ) ;
#54621=DIRECTION ( 'NONE',  ( 0.000000000000000000, 1.000000000000000000, 0.000000000000000000 ) ) ;
#54622=CIRCLE ( 'NONE', #50429, 0.06509327318403745899 ) ;
#54623=LINE ( 'NONE', #74288, #16184 ) ;
#54624=CARTESIAN_POINT ( 'NONE',  ( -3.350000000000028955, 2.500000000000000000, 2.265063509461097357 ) ) ;
#54625=CARTESIAN_POINT ( 'NONE',  ( -10.85000000000000142, 12.50000000000000000, -7.188010851410850499 ) ) ;
#54626=AXIS2_PLACEMENT_3D ( 'NONE', #112963, #92033, #13463 ) ;
#54627=CARTESIAN_POINT ( 'NONE',  ( -8.950000000000008171, 2.500000000000000000, -2.411473670974877859 ) ) ;
#54628=AXIS2_PLACEMENT_3D ( 'NONE', #92058, #2371, #73701 ) ;
#54629=EDGE_LOOP ( 'NONE', ( #40492, #32569 ) ) ;
#54630=CARTESIAN_POINT ( 'NONE',  ( 13.29999999999990301, 2.500000000000000000, -4.330127018922201643 ) ) ;
#54631=VERTEX_POINT ( 'NONE', #87442 ) ;
#54632=CARTESIAN_POINT ( 'NONE',  ( 17.50000000000000000, 2.500000000000000000, -3.999999999999996447 ) ) ;
#54633=VERTEX_POINT ( 'NONE', #37717 ) ;
#54634=DIRECTION ( 'NONE',  ( -0.000000000000000000, 1.000000000000000000, -0.000000000000000000 ) ) ;
#54635=CONICAL_SURFACE ( 'NONE', #35870, 0.1000000000000002554, 0.003490658503988666988 ) ;
#54636=CIRCLE ( 'NONE', #125644, 0.09999999999999999167 ) ;
#54637=DIRECTION ( 'NONE',  ( 0.000000000000000000, -0.000000000000000000, 1.000000000000000000 ) ) ;
#54638=CARTESIAN_POINT ( 'NONE',  ( 6.249999999999967137, 12.50000000000000000, -2.230156782645139391 ) ) ;
#54639=CARTESIAN_POINT ( 'NONE',  ( 0.7999999999999548583, 2.500000000000000000, 4.330127018922196314 ) ) ;
#54640=EDGE_LOOP ( 'NONE', ( #48446, #61783, #112505, #68612 ) ) ;
#54641=CARTESIAN_POINT ( 'NONE',  ( 1.649999999999948841, 12.50000000000000000, 6.495190528383297135 ) ) ;
#54642=DIRECTION ( 'NONE',  ( 0.000000000000000000, 0.000000000000000000, 1.000000000000000000 ) ) ;
#54643=VERTEX_POINT ( 'NONE', #77622 ) ;
#54644=ORIENTED_EDGE ( 'NONE', *, *, #29269, .F. ) ;
#54645=ORIENTED_EDGE ( 'NONE', *, *, #109409, .T. ) ;
#54646=DIRECTION ( 'NONE',  ( 0.000000000000000000, 1.000000000000000000, 0.000000000000000000 ) ) ;
#54647=FACE_OUTER_BOUND ( 'NONE', #44069, .T. ) ;
#54649=CARTESIAN_POINT ( 'NONE',  ( 13.14999999999990088, 2.500000000000000000, 2.511473670974873507 ) ) ;
#54650=CARTESIAN_POINT ( 'NONE',  ( 11.84999999999990727, 12.50000000000000000, -1.818653347947326138 ) ) ;
#54651=ADVANCED_FACE ( 'NONE', ( #18710 ), #55019, .T. ) ;
#54652=DIRECTION ( 'NONE',  ( -0.000000000000000000, 1.000000000000000000, -0.000000000000000000 ) ) ;
#54653=AXIS2_PLACEMENT_3D ( 'NONE', #75116, #85574, #36499 ) ;
#54654=VECTOR ( 'NONE', #76064, 1000.000000000000000 ) ;
#54655=ORIENTED_EDGE ( 'NONE', *, *, #57239, .T. ) ;
#54656=DIRECTION ( 'NONE',  ( 0.000000000000000000, -0.000000000000000000, 1.000000000000000000 ) ) ;
#54657=CIRCLE ( 'NONE', #96508, 0.1000000000000000472 ) ;
#54658=VECTOR ( 'NONE', #4355, 1000.000000000000000 ) ;
#54659=EDGE_LOOP ( 'NONE', ( #128457, #95523, #129024, #107755 ) ) ;
#54661=EDGE_CURVE ( 'NONE', #9617, #5036, #60872, .T. ) ;
#54662=LINE ( 'NONE', #23943, #18301 ) ;
#54664=DIRECTION ( 'NONE',  ( -4.274815082592931898E-19, -0.9999939076577903929, -0.003490651415223739937 ) ) ;
#54665=EDGE_LOOP ( 'NONE', ( #53652, #73922 ) ) ;
#54666=DIRECTION ( 'NONE',  ( 0.000000000000000000, -0.9999939076577903929, 0.003490651415223739937 ) ) ;
#54667=LINE ( 'NONE', #95269, #104018 ) ;
#54668=ORIENTED_EDGE ( 'NONE', *, *, #127741, .F. ) ;
#54669=DIRECTION ( 'NONE',  ( -0.000000000000000000, -1.000000000000000000, -0.000000000000000000 ) ) ;
#54670=ORIENTED_EDGE ( 'NONE', *, *, #90962, .F. ) ;
#54671=ORIENTED_EDGE ( 'NONE', *, *, #52192, .T. ) ;
#54672=CARTESIAN_POINT ( 'NONE',  ( -11.24999999999996270, 2.500000000000000000, 6.395190528383296602 ) ) ;
#54673=ORIENTED_EDGE ( 'NONE', *, *, #123563, .F. ) ;
#54674=CARTESIAN_POINT ( 'NONE',  ( 2.299999999999949640, 2.500000000000000000, -0.4464101615137782142 ) ) ;
#54675=DIRECTION ( 'NONE',  ( 0.000000000000000000, 1.000000000000000000, 0.000000000000000000 ) ) ;
#54676=DIRECTION ( 'NONE',  ( 0.000000000000000000, 1.000000000000000000, 0.000000000000000000 ) ) ;
#54677=AXIS2_PLACEMENT_3D ( 'NONE', #97337, #7004, #17470 ) ;
#54678=VERTEX_POINT ( 'NONE', #120442 ) ;
#54679=AXIS2_PLACEMENT_3D ( 'NONE', #35513, #125793, #95717 ) ;
#54680=EDGE_CURVE ( 'NONE', #91293, #64031, #128198, .T. ) ;
#54681=FACE_BOUND ( 'NONE', #68437, .T. ) ;
#54682=CARTESIAN_POINT ( 'NONE',  ( -3.550000000000028688, 2.500000000000000000, 6.841600689897072485 ) ) ;
#54683=CARTESIAN_POINT ( 'NONE',  ( -8.749999999999975131, 2.500000000000000000, 2.065063509461097624 ) ) ;
#54684=ORIENTED_EDGE ( 'NONE', *, *, #31293, .F. ) ;
#54685=CARTESIAN_POINT ( 'NONE',  ( -5.200000000000022382, 12.50000000000000000, 4.676537180435972552 ) ) ;
#54687=AXIS2_PLACEMENT_3D ( 'NONE', #88996, #69336, #9784 ) ;
#54688=EDGE_CURVE ( 'NONE', #121723, #26124, #62182, .T. ) ;
#54689=ORIENTED_EDGE ( 'NONE', *, *, #56393, .F. ) ;
#54690=CIRCLE ( 'NONE', #94507, 0.06509327318403745899 ) ;
#54691=CONICAL_SURFACE ( 'NONE', #127876, 0.1000000000000002554, 0.003490658503988666988 ) ;
#54692=AXIS2_PLACEMENT_3D ( 'NONE', #20713, #121470, #119538 ) ;
#54693=ORIENTED_EDGE ( 'NONE', *, *, #41777, .F. ) ;
#54694=ORIENTED_EDGE ( 'NONE', *, *, #36594, .F. ) ;
#54695=DIRECTION ( 'NONE',  ( -0.000000000000000000, -1.000000000000000000, -0.000000000000000000 ) ) ;
#54696=DIRECTION ( 'NONE',  ( 0.000000000000000000, 0.000000000000000000, -1.000000000000000000 ) ) ;
#54697=EDGE_CURVE ( 'NONE', #60586, #101827, #100161, .T. ) ;
#54698=EDGE_CURVE ( 'NONE', #101462, #1863, #63440, .T. ) ;
#54699=DIRECTION ( 'NONE',  ( 0.000000000000000000, -0.000000000000000000, 1.000000000000000000 ) ) ;
#54700=EDGE_CURVE ( 'NONE', #79310, #57270, #6972, .T. ) ;
#54701=FACE_BOUND ( 'NONE', #121611, .T. ) ;
#54702=VERTEX_POINT ( 'NONE', #3249 ) ;
#54703=EDGE_CURVE ( 'NONE', #118649, #80208, #9050, .T. ) ;
#54705=EDGE_CURVE ( 'NONE', #34772, #86996, #1939, .T. ) ;
#54706=CARTESIAN_POINT ( 'NONE',  ( 2.499999999999983569, 2.500000000000000000, -2.276824562219559311E-15 ) ) ;
#54707=CARTESIAN_POINT ( 'NONE',  ( 14.99999999999989342, 2.500000000000000000, -0.5928203230275541635 ) ) ;
#54708=AXIS2_PLACEMENT_3D ( 'NONE', #37655, #59239, #117449 ) ;
#54709=DIRECTION ( 'NONE',  ( -0.000000000000000000, 1.000000000000000000, -0.000000000000000000 ) ) ;
#54710=CONICAL_SURFACE ( 'NONE', #69477, 0.1000000000000002554, 0.003490658503988666988 ) ;
#54711=CARTESIAN_POINT ( 'NONE',  ( 4.149999999999941735, 2.500000000000000000, -1.472243186433550122 ) ) ;
#54712=AXIS2_PLACEMENT_3D ( 'NONE', #5366, #123847, #43390 ) ;
#54713=CIRCLE ( 'NONE', #38301, 0.1000000000000002554 ) ;
#54714=CARTESIAN_POINT ( 'NONE',  ( -4.600000000000028066, 2.500000000000000000, -5.022947341949754119 ) ) ;
#54715=FACE_OUTER_BOUND ( 'NONE', #38833, .T. ) ;
#54716=EDGE_CURVE ( 'NONE', #39745, #127685, #42532, .T. ) ;
#54717=CARTESIAN_POINT ( 'NONE',  ( -3.750000000000029310, 12.50000000000000000, -7.188010851410854052 ) ) ;
#54718=AXIS2_PLACEMENT_3D ( 'NONE', #100445, #71626, #42172 ) ;
#54719=EDGE_CURVE ( 'NONE', #68377, #115059, #80163, .T. ) ;
#54720=EDGE_CURVE ( 'NONE', #82397, #19127, #90720, .T. ) ;
#54721=DIRECTION ( 'NONE',  ( 0.000000000000000000, -0.9999939076577903929, 0.003490651415223739937 ) ) ;
#54722=VERTEX_POINT ( 'NONE', #50403 ) ;
#54723=AXIS2_PLACEMENT_3D ( 'NONE', #15111, #66169, #104791 ) ;
#54724=ORIENTED_EDGE ( 'NONE', *, *, #66419, .F. ) ;
#54725=EDGE_LOOP ( 'NONE', ( #13880, #11275 ) ) ;
#54726=EDGE_LOOP ( 'NONE', ( #22395, #28718 ) ) ;
#54727=EDGE_LOOP ( 'NONE', ( #79931, #67611, #98435, #123352 ) ) ;
#54728=DIRECTION ( 'NONE',  ( 0.000000000000000000, 1.000000000000000000, 0.000000000000000000 ) ) ;
#54729=DIRECTION ( 'NONE',  ( 0.000000000000000000, 0.000000000000000000, 1.000000000000000000 ) ) ;
#54730=ORIENTED_EDGE ( 'NONE', *, *, #28186, .T. ) ;
#54731=FACE_BOUND ( 'NONE', #60898, .T. ) ;
#54732=CARTESIAN_POINT ( 'NONE',  ( 1.649999999999951505, 2.500000000000000000, -1.372243186433550033 ) ) ;
#54733=CARTESIAN_POINT ( 'NONE',  ( -0.2000000000000339284, 2.500000000000000000, -0.4464101615137759382 ) ) ;
#54734=ORIENTED_EDGE ( 'NONE', *, *, #62884, .T. ) ;
#54735=FACE_OUTER_BOUND ( 'NONE', #87894, .T. ) ;
#54736=CARTESIAN_POINT ( 'NONE',  ( -10.45000000000000107, 2.500000000000000000, 2.265063509461097357 ) ) ;
#54737=DIRECTION ( 'NONE',  ( 0.000000000000000000, 0.000000000000000000, 1.000000000000000000 ) ) ;
#54738=EDGE_LOOP ( 'NONE', ( #47960, #106395 ) ) ;
#54739=DIRECTION ( 'NONE',  ( 0.000000000000000000, 0.000000000000000000, 1.000000000000000000 ) ) ;
#54740=ORIENTED_EDGE ( 'NONE', *, *, #39213, .T. ) ;
#54741=ORIENTED_EDGE ( 'NONE', *, *, #113666, .F. ) ;
#54742=VECTOR ( 'NONE', #14769, 1000.000000000000000 ) ;
#54743=ORIENTED_EDGE ( 'NONE', *, *, #49233, .T. ) ;
#54744=CIRCLE ( 'NONE', #23560, 0.1000000000000002554 ) ;
#54745=LINE ( 'NONE', #64575, #6670 ) ;
#54746=AXIS2_PLACEMENT_3D ( 'NONE', #100836, #91036, #79924 ) ;
#54747=FACE_OUTER_BOUND ( 'NONE', #1036, .T. ) ;
#54748=CARTESIAN_POINT ( 'NONE',  ( -3.642919299551294898E-14, 12.50000000000000000, 0.6928203230275518099 ) ) ;
#54749=ORIENTED_EDGE ( 'NONE', *, *, #67891, .T. ) ;
#54750=CARTESIAN_POINT ( 'NONE',  ( 2.500000000000002220, 2.499999999999998668, -9.000000000000000000 ) ) ;
#54751=CARTESIAN_POINT ( 'NONE',  ( 1.649999999999951950, 2.500000000000000000, -7.088010851410853519 ) ) ;
#54752=CONICAL_SURFACE ( 'NONE', #127928, 0.1000000000000000472, 0.003490658503988666988 ) ;
#54753=AXIS2_PLACEMENT_3D ( 'NONE', #14411, #54346, #101522 ) ;
#54754=CIRCLE ( 'NONE', #73536, 0.06509327318403745899 ) ;
#54755=DIRECTION ( 'NONE',  ( -0.000000000000000000, 1.000000000000000000, -0.000000000000000000 ) ) ;
#54757=DIRECTION ( 'NONE',  ( 0.000000000000000000, -0.9999939076577903929, 0.003490651415223739937 ) ) ;
#54758=VERTEX_POINT ( 'NONE', #110613 ) ;
#54759=AXIS2_PLACEMENT_3D ( 'NONE', #60590, #1635, #120137 ) ;
#54760=CIRCLE ( 'NONE', #71490, 0.06509327318403743123 ) ;
#54761=DIRECTION ( 'NONE',  ( 0.000000000000000000, 1.000000000000000000, 0.000000000000000000 ) ) ;
#54762=ADVANCED_FACE ( 'NONE', ( #11112 ), #51029, .T. ) ;
#54763=ORIENTED_EDGE ( 'NONE', *, *, #105893, .F. ) ;
#54764=DIRECTION ( 'NONE',  ( 0.000000000000000000, 0.000000000000000000, 1.000000000000000000 ) ) ;
#54765=CONICAL_SURFACE ( 'NONE', #29649, 0.09999999999999982514, 0.003490658503988666988 ) ;
#54766=EDGE_CURVE ( 'NONE', #38253, #112855, #53072, .T. ) ;
#54767=EDGE_LOOP ( 'NONE', ( #64574, #35749, #103685, #46292 ) ) ;
#54768=EDGE_CURVE ( 'NONE', #73062, #66361, #73999, .T. ) ;
#54769=ORIENTED_EDGE ( 'NONE', *, *, #54149, .F. ) ;
#54770=CARTESIAN_POINT ( 'NONE',  ( 3.299999999999944755, 12.50000000000000000, -4.395220292106239768 ) ) ;
#54771=DIRECTION ( 'NONE',  ( -0.000000000000000000, -1.000000000000000000, -0.000000000000000000 ) ) ;
#54772=DIRECTION ( 'NONE',  ( 0.000000000000000000, 0.000000000000000000, 1.000000000000000000 ) ) ;
#54773=FACE_OUTER_BOUND ( 'NONE', #65478, .T. ) ;
#54774=LINE ( 'NONE', #94068, #34940 ) ;
#54775=ORIENTED_EDGE ( 'NONE', *, *, #27785, .F. ) ;
#54776=EDGE_CURVE ( 'NONE', #25337, #22838, #128296, .T. ) ;
#54777=VERTEX_POINT ( 'NONE', #102090 ) ;
#54778=PLANE ( 'NONE',  #85249 ) ;
#54779=DIRECTION ( 'NONE',  ( -0.000000000000000000, -1.000000000000000000, -0.000000000000000000 ) ) ;
#54780=FACE_OUTER_BOUND ( 'NONE', #56431, .T. ) ;
#54781=ORIENTED_EDGE ( 'NONE', *, *, #15050, .F. ) ;
#54783=DIRECTION ( 'NONE',  ( -0.000000000000000000, -1.000000000000000000, -0.000000000000000000 ) ) ;
#54784=AXIS2_PLACEMENT_3D ( 'NONE', #71101, #10858, #110376 ) ;
#54785=ORIENTED_EDGE ( 'NONE', *, *, #36832, .T. ) ;
#54786=CARTESIAN_POINT ( 'NONE',  ( 6.049999999999932321, 12.50000000000000000, -1.753560074763288679 ) ) ;
#54787=CARTESIAN_POINT ( 'NONE',  ( -0.6500000000000394351, 2.500000000000000000, 2.411473670974873862 ) ) ;
#54788=ORIENTED_EDGE ( 'NONE', *, *, #95656, .T. ) ;
#54789=DIRECTION ( 'NONE',  ( 0.000000000000000000, 1.000000000000000000, 0.000000000000000000 ) ) ;
#54790=DIRECTION ( 'NONE',  ( 0.000000000000000000, 0.000000000000000000, 1.000000000000000000 ) ) ;
#54791=CARTESIAN_POINT ( 'NONE',  ( 5.649999999999932854, 2.500000000000000000, 2.511473670974873507 ) ) ;
#54792=EDGE_CURVE ( 'NONE', #111183, #84285, #38420, .T. ) ;
#54793=CARTESIAN_POINT ( 'NONE',  ( 9.799999999999915445, 2.500000000000000000, -4.676537180435977881 ) ) ;
#54794=AXIS2_PLACEMENT_3D ( 'NONE', #84967, #7031, #54853 ) ;
#54795=ORIENTED_EDGE ( 'NONE', *, *, #41031, .T. ) ;
#54796=AXIS2_PLACEMENT_3D ( 'NONE', #1659, #10205, #2295 ) ;
#54797=AXIS2_PLACEMENT_3D ( 'NONE', #8598, #48556, #79317 ) ;
#54798=PLANE ( 'NONE',  #65446 ) ;
#54799=AXIS2_PLACEMENT_3D ( 'NONE', #122778, #4264, #33749 ) ;
#54800=DIRECTION ( 'NONE',  ( 0.000000000000000000, 0.000000000000000000, 1.000000000000000000 ) ) ;
#54801=VERTEX_POINT ( 'NONE', #73268 ) ;
#54802=ORIENTED_EDGE ( 'NONE', *, *, #107155, .T. ) ;
#54804=DIRECTION ( 'NONE',  ( 0.000000000000000000, 1.000000000000000000, 0.000000000000000000 ) ) ;
#54805=CARTESIAN_POINT ( 'NONE',  ( -10.20000000000000462, 2.500000000000000000, -4.676537180435973440 ) ) ;
#54806=LINE ( 'NONE', #56098, #51118 ) ;
#54807=DIRECTION ( 'NONE',  ( -4.274815082592931898E-19, -0.9999939076577903929, -0.003490651415223739937 ) ) ;
#54808=CIRCLE ( 'NONE', #36043, 0.1000000000000000472 ) ;
#54809=FACE_OUTER_BOUND ( 'NONE', #1360, .T. ) ;
#54810=EDGE_CURVE ( 'NONE', #43068, #125419, #23826, .T. ) ;
#54811=AXIS2_PLACEMENT_3D ( 'NONE', #47340, #85315, #55850 ) ;
#54812=DIRECTION ( 'NONE',  ( -0.000000000000000000, -1.000000000000000000, -0.000000000000000000 ) ) ;
#54813=CARTESIAN_POINT ( 'NONE',  ( -9.150000000000005684, 2.500000000000000000, 5.802370205355744659 ) ) ;
#54814=CIRCLE ( 'NONE', #29782, 0.1000000000000002554 ) ;
#54815=CARTESIAN_POINT ( 'NONE',  ( 8.949999999999919353, 2.500000000000000000, -6.148780366869526226 ) ) ;
#54817=LINE ( 'NONE', #43109, #85636 ) ;
#54818=ORIENTED_EDGE ( 'NONE', *, *, #30090, .F. ) ;
#54820=CONICAL_SURFACE ( 'NONE', #123868, 0.1000000000000002554, 0.003490658503988666988 ) ;
#54821=ORIENTED_EDGE ( 'NONE', *, *, #120857, .T. ) ;
#54822=ORIENTED_EDGE ( 'NONE', *, *, #8272, .F. ) ;
#54823=EDGE_CURVE ( 'NONE', #46586, #43896, #122027, .T. ) ;
#54824=CARTESIAN_POINT ( 'NONE',  ( 10.39999999999991154, 2.500000000000000000, 3.737306695894644371 ) ) ;
#54825=DIRECTION ( 'NONE',  ( -0.000000000000000000, -1.000000000000000000, -0.000000000000000000 ) ) ;
#54826=DIRECTION ( 'NONE',  ( 0.000000000000000000, 0.000000000000000000, -1.000000000000000000 ) ) ;
#54827=ORIENTED_EDGE ( 'NONE', *, *, #97464, .T. ) ;
#54828=CARTESIAN_POINT ( 'NONE',  ( -9.350000000000006750, 2.500000000000000000, -1.918653347947325782 ) ) ;
#54829=CARTESIAN_POINT ( 'NONE',  ( -4.150000000000027889, 2.500000000000000000, -7.188010851410854052 ) ) ;
#54830=CARTESIAN_POINT ( 'NONE',  ( 9.999999999999914735, 2.500000000000000000, 0.7928203230275495672 ) ) ;
#54831=EDGE_LOOP ( 'NONE', ( #91848, #30739 ) ) ;
#54832=CARTESIAN_POINT ( 'NONE',  ( 9.999999999999912959, 2.500000000000000000, 3.537306695894645081 ) ) ;
#54833=ORIENTED_EDGE ( 'NONE', *, *, #12725, .T. ) ;
#54834=VERTEX_POINT ( 'NONE', #2575 ) ;
#54835=VERTEX_POINT ( 'NONE', #72639 ) ;
#54836=CIRCLE ( 'NONE', #79893, 0.06509327318403741736 ) ;
#54837=VERTEX_POINT ( 'NONE', #4495 ) ;
#54838=CARTESIAN_POINT ( 'NONE',  ( -2.100000000000034284, 12.50000000000000000, -4.330127018922201643 ) ) ;
#54839=AXIS2_PLACEMENT_3D ( 'NONE', #104705, #94901, #5219 ) ;
#54840=FACE_OUTER_BOUND ( 'NONE', #25015, .T. ) ;
#54841=LINE ( 'NONE', #35236, #65077 ) ;
#54842=CARTESIAN_POINT ( 'NONE',  ( -5.650000000000023448, 2.500000000000000000, -6.148780366869526226 ) ) ;
#54843=ORIENTED_EDGE ( 'NONE', *, *, #94665, .T. ) ;
#54844=CIRCLE ( 'NONE', #44396, 0.1000000000000002554 ) ;
#54845=EDGE_CURVE ( 'NONE', #67610, #50039, #96128, .T. ) ;
#54846=LINE ( 'NONE', #55515, #14707 ) ;
#54847=AXIS2_PLACEMENT_3D ( 'NONE', #104359, #25796, #64428 ) ;
#54848=ORIENTED_EDGE ( 'NONE', *, *, #16120, .T. ) ;
#54849=FACE_OUTER_BOUND ( 'NONE', #23456, .T. ) ;
#54850=CARTESIAN_POINT ( 'NONE',  ( -0.2000000000000347888, 12.50000000000000000, 0.3464101615137758494 ) ) ;
#54851=CONICAL_SURFACE ( 'NONE', #105027, 0.09999999999999982514, 0.003490658503988666988 ) ;
#54853=DIRECTION ( 'NONE',  ( 0.000000000000000000, 0.000000000000000000, 1.000000000000000000 ) ) ;
#54854=CIRCLE ( 'NONE', #86148, 0.1000000000000002554 ) ;
#54855=ADVANCED_FACE ( 'NONE', ( #3879 ), #61394, .T. ) ;
#54856=ORIENTED_EDGE ( 'NONE', *, *, #114871, .T. ) ;
#54858=ORIENTED_EDGE ( 'NONE', *, *, #60972, .F. ) ;
#54859=DIRECTION ( 'NONE',  ( 0.000000000000000000, 0.000000000000000000, 1.000000000000000000 ) ) ;
#54860=CARTESIAN_POINT ( 'NONE',  ( -13.34999999999999076, 12.50000000000000000, 2.792790559304615616 ) ) ;
#54861=EDGE_CURVE ( 'NONE', #9027, #126067, #24817, .T. ) ;
#54862=ADVANCED_FACE ( 'NONE', ( #114479 ), #30104, .T. ) ;
#54863=DIRECTION ( 'NONE',  ( -0.000000000000000000, -1.000000000000000000, -0.000000000000000000 ) ) ;
#54864=EDGE_CURVE ( 'NONE', #115574, #24359, #92787, .T. ) ;
#54865=FACE_BOUND ( 'NONE', #78429, .T. ) ;
#54866=EDGE_CURVE ( 'NONE', #88265, #6869, #40573, .T. ) ;
#54867=CARTESIAN_POINT ( 'NONE',  ( 1.849999999999950129, 12.50000000000000000, -6.841600689897078702 ) ) ;
#54868=CARTESIAN_POINT ( 'NONE',  ( -9.800000000000007816, 2.500000000000000000, -3.983716857408421852 ) ) ;
#54869=DIRECTION ( 'NONE',  ( 0.000000000000000000, 1.000000000000000000, 0.000000000000000000 ) ) ;
#54870=AXIS2_PLACEMENT_3D ( 'NONE', #11546, #82238, #50841 ) ;
#54871=EDGE_CURVE ( 'NONE', #51072, #98382, #19620, .T. ) ;
#54873=EDGE_CURVE ( 'NONE', #109616, #58961, #93560, .T. ) ;
#54874=CARTESIAN_POINT ( 'NONE',  ( 8.099999999999923261, 2.500000000000000000, 4.676537180435972552 ) ) ;
#54875=EDGE_CURVE ( 'NONE', #67325, #114219, #15387, .T. ) ;
#54876=CARTESIAN_POINT ( 'NONE',  ( -4.550000000000022915, 12.50000000000000000, -2.165063509461101710 ) ) ;
#54877=EDGE_LOOP ( 'NONE', ( #106114, #98700 ) ) ;
#54878=AXIS2_PLACEMENT_3D ( 'NONE', #99128, #98455, #8790 ) ;
#54879=EDGE_CURVE ( 'NONE', #12234, #70177, #99042, .T. ) ;
#54880=CIRCLE ( 'NONE', #25636, 0.06509327318403745899 ) ;
#54881=EDGE_CURVE ( 'NONE', #73196, #61030, #88567, .T. ) ;
#54882=DIRECTION ( 'NONE',  ( 0.000000000000000000, 0.000000000000000000, 1.000000000000000000 ) ) ;
#54883=ORIENTED_EDGE ( 'NONE', *, *, #48116, .T. ) ;
#54884=EDGE_LOOP ( 'NONE', ( #122187, #94170 ) ) ;
#54885=VERTEX_POINT ( 'NONE', #45754 ) ;
#54886=VERTEX_POINT ( 'NONE', #35922 ) ;
#54887=DIRECTION ( 'NONE',  ( 0.000000000000000000, 1.000000000000000000, 0.000000000000000000 ) ) ;
#54888=FACE_BOUND ( 'NONE', #102515, .T. ) ;
#54889=AXIS2_PLACEMENT_3D ( 'NONE', #107011, #58591, #98484 ) ;
#54890=EDGE_CURVE ( 'NONE', #2948, #29851, #25876, .T. ) ;
#54891=DIRECTION ( 'NONE',  ( 0.000000000000000000, 0.000000000000000000, 1.000000000000000000 ) ) ;
#54892=CIRCLE ( 'NONE', #52744, 0.06509327318403745899 ) ;
#54893=CONICAL_SURFACE ( 'NONE', #75819, 0.1000000000000002554, 0.003490658503988666988 ) ;
#54894=CIRCLE ( 'NONE', #38184, 0.09999999999999982514 ) ;
#54896=CARTESIAN_POINT ( 'NONE',  ( 26.75237029038848391, 2.962322469582319151, 2.722363819593919931 ) ) ;
#54897=DIRECTION ( 'NONE',  ( 0.000000000000000000, 1.000000000000000000, 0.000000000000000000 ) ) ;
#54898=ORIENTED_EDGE ( 'NONE', *, *, #91472, .T. ) ;
#54899=CIRCLE ( 'NONE', #117574, 0.06509327318403745899 ) ;
#54900=DIRECTION ( 'NONE',  ( 0.000000000000000000, 1.000000000000000000, 0.000000000000000000 ) ) ;
#54901=DIRECTION ( 'NONE',  ( 0.000000000000000000, 1.000000000000000000, 0.000000000000000000 ) ) ;
#54902=VECTOR ( 'NONE', #128984, 1000.000000000000000 ) ;
#54903=CIRCLE ( 'NONE', #94607, 0.06509327318403745899 ) ;
#54904=AXIS2_PLACEMENT_3D ( 'NONE', #123682, #53043, #15664 ) ;
#54905=CONICAL_SURFACE ( 'NONE', #128085, 0.09999999999999982514, 0.003490658503988666988 ) ;
#54906=ORIENTED_EDGE ( 'NONE', *, *, #2797, .F. ) ;
#54907=DIRECTION ( 'NONE',  ( -0.000000000000000000, -1.000000000000000000, -0.000000000000000000 ) ) ;
#54908=DIRECTION ( 'NONE',  ( -4.274815082592931898E-19, -0.9999939076577903929, -0.003490651415223739937 ) ) ;
#54909=EDGE_LOOP ( 'NONE', ( #62657, #49461, #36248, #73100 ) ) ;
#54910=CARTESIAN_POINT ( 'NONE',  ( -3.550000000000028244, 2.500000000000000000, 2.411473670974873862 ) ) ;
#54911=CIRCLE ( 'NONE', #627, 0.1000000000000000472 ) ;
#54912=CARTESIAN_POINT ( 'NONE',  ( 6.649999999999929301, 2.500000000000000000, -2.165063509461101710 ) ) ;
#54913=DIRECTION ( 'NONE',  ( -0.000000000000000000, -1.000000000000000000, -0.000000000000000000 ) ) ;
#54914=ORIENTED_EDGE ( 'NONE', *, *, #15268, .T. ) ;
#54915=ORIENTED_EDGE ( 'NONE', *, *, #124636, .F. ) ;
#54916=DIRECTION ( 'NONE',  ( -0.000000000000000000, -1.000000000000000000, -0.000000000000000000 ) ) ;
#54917=ORIENTED_EDGE ( 'NONE', *, *, #126105, .T. ) ;
#54918=CARTESIAN_POINT ( 'NONE',  ( 10.59999999999990905, 12.50000000000000000, -4.048810130592463530 ) ) ;
#54919=DIRECTION ( 'NONE',  ( 0.000000000000000000, 1.000000000000000000, 0.000000000000000000 ) ) ;
#54920=EDGE_CURVE ( 'NONE', #16529, #95073, #11295, .T. ) ;
#54921=VERTEX_POINT ( 'NONE', #105955 ) ;
#54923=ADVANCED_FACE ( 'NONE', ( #14958 ), #46815, .T. ) ;
#54924=FACE_OUTER_BOUND ( 'NONE', #66739, .T. ) ;
#54925=PLANE ( 'NONE',  #17260 ) ;
#54926=AXIS2_PLACEMENT_3D ( 'NONE', #91663, #111963, #92966 ) ;
#54927=CARTESIAN_POINT ( 'NONE',  ( 12.89999999999990266, 12.50000000000000000, -3.637306695894650055 ) ) ;
#54928=VECTOR ( 'NONE', #36667, 1000.000000000000000 ) ;
#54929=LINE ( 'NONE', #35313, #59897 ) ;
#54930=EDGE_CURVE ( 'NONE', #32336, #70678, #25436, .T. ) ;
#54931=ORIENTED_EDGE ( 'NONE', *, *, #36495, .T. ) ;
#54932=VERTEX_POINT ( 'NONE', #54910 ) ;
#54933=CARTESIAN_POINT ( 'NONE',  ( 1.849999999999949019, 12.50000000000000000, 6.906693963081109722 ) ) ;
#54934=EDGE_CURVE ( 'NONE', #25178, #13086, #64095, .T. ) ;
#54935=AXIS2_PLACEMENT_3D ( 'NONE', #85477, #125405, #26565 ) ;
#54936=LINE ( 'NONE', #64756, #114227 ) ;
#54938=CIRCLE ( 'NONE', #128111, 0.1000000000000000472 ) ;
#54939=CARTESIAN_POINT ( 'NONE',  ( -7.900000000000014566, 2.500000000000000000, 0.09999999999999772959 ) ) ;
#54940=ORIENTED_EDGE ( 'NONE', *, *, #36976, .F. ) ;
#54941=ORIENTED_EDGE ( 'NONE', *, *, #20437, .F. ) ;
#54942=ORIENTED_EDGE ( 'NONE', *, *, #108103, .T. ) ;
#54943=CARTESIAN_POINT ( 'NONE',  ( -14.99999999999998401, 2.500000000000000000, 0.6928203230275518099 ) ) ;
#54944=CARTESIAN_POINT ( 'NONE',  ( -1.450000000000035927, 2.500000000000000000, -6.148780366869526226 ) ) ;
#54945=VECTOR ( 'NONE', #13131, 1000.000000000000000 ) ;
#54946=CIRCLE ( 'NONE', #57096, 0.1000000000000000472 ) ;
#54947=DIRECTION ( 'NONE',  ( 0.000000000000000000, -0.9999939076577903929, 0.003490651415223739937 ) ) ;
#54948=AXIS2_PLACEMENT_3D ( 'NONE', #3637, #62576, #43587 ) ;
#54950=CARTESIAN_POINT ( 'NONE',  ( 10.84999999999990905, 2.500000000000000000, 2.165063509461097713 ) ) ;
#54951=DIRECTION ( 'NONE',  ( 0.000000000000000000, -0.9999939076577903929, 0.003490651415223739937 ) ) ;
#54953=VECTOR ( 'NONE', #119320, 1000.000000000000000 ) ;
#54954=LINE ( 'NONE', #43230, #1096 ) ;
#54955=LINE ( 'NONE', #35333, #84362 ) ;
#54956=CONICAL_SURFACE ( 'NONE', #86340, 0.09999999999999982514, 0.003490658503988666988 ) ;
#54957=DIRECTION ( 'NONE',  ( 0.000000000000000000, 0.000000000000000000, -1.000000000000000000 ) ) ;
#54958=AXIS2_PLACEMENT_3D ( 'NONE', #97962, #19393, #119530 ) ;
#54959=VERTEX_POINT ( 'NONE', #94848 ) ;
#54960=CARTESIAN_POINT ( 'NONE',  ( 13.29999999999989946, 12.50000000000000000, 0.06509327318403504425 ) ) ;
#54961=EDGE_LOOP ( 'NONE', ( #25009, #43607 ) ) ;
#54962=ORIENTED_EDGE ( 'NONE', *, *, #73783, .F. ) ;
#54963=DIRECTION ( 'NONE',  ( 0.000000000000000000, 0.000000000000000000, -1.000000000000000000 ) ) ;
#54964=CARTESIAN_POINT ( 'NONE',  ( 8.949999999999917577, 2.500000000000000000, -2.611473670974877592 ) ) ;
#54965=FACE_OUTER_BOUND ( 'NONE', #40250, .T. ) ;
#54966=CONICAL_SURFACE ( 'NONE', #128142, 0.1000000000000002554, 0.003490658503988666988 ) ;
#54967=EDGE_CURVE ( 'NONE', #37345, #25872, #65583, .T. ) ;
#54968=DIRECTION ( 'NONE',  ( 0.000000000000000000, 0.000000000000000000, 1.000000000000000000 ) ) ;
#54969=CARTESIAN_POINT ( 'NONE',  ( 7.699999999999925571, 2.500000000000000000, -4.776537180435978414 ) ) ;
#54970=DIRECTION ( 'NONE',  ( 0.000000000000000000, 0.000000000000000000, 1.000000000000000000 ) ) ;
#54971=LINE ( 'NONE', #112620, #32182 ) ;
#54973=DIRECTION ( 'NONE',  ( 0.000000000000000000, 1.000000000000000000, 0.000000000000000000 ) ) ;
#54974=CIRCLE ( 'NONE', #15243, 0.1000000000000002554 ) ;
#54975=DIRECTION ( 'NONE',  ( 0.000000000000000000, 0.000000000000000000, 1.000000000000000000 ) ) ;
#54976=ORIENTED_EDGE ( 'NONE', *, *, #50731, .F. ) ;
#54977=AXIS2_PLACEMENT_3D ( 'NONE', #7240, #68753, #128350 ) ;
#54978=ORIENTED_EDGE ( 'NONE', *, *, #37624, .F. ) ;
#54979=EDGE_LOOP ( 'NONE', ( #64572, #88523 ) ) ;
#54980=ADVANCED_FACE ( 'NONE', ( #124309 ), #85664, .T. ) ;
#54981=ADVANCED_FACE ( 'NONE', ( #8384 ), #4923, .T. ) ;
#54982=EDGE_LOOP ( 'NONE', ( #118965, #5979 ) ) ;
#54983=AXIS2_PLACEMENT_3D ( 'NONE', #947, #4620, #43944 ) ;
#54984=CARTESIAN_POINT ( 'NONE',  ( -5.000000000000024869, 2.500000000000000000, -5.022947341949754119 ) ) ;
#54985=DIRECTION ( 'NONE',  ( 0.000000000000000000, 0.000000000000000000, 1.000000000000000000 ) ) ;
#54986=AXIS2_PLACEMENT_3D ( 'NONE', #87635, #79762, #100054 ) ;
#54987=AXIS2_PLACEMENT_3D ( 'NONE', #18378, #70066, #121093 ) ;
#54988=CARTESIAN_POINT ( 'NONE',  ( 16.55763163376620994, 0.1615157349276458432, -6.093150851882356278 ) ) ;
#54989=AXIS2_PLACEMENT_3D ( 'NONE', #40045, #79960, #120536 ) ;
#54990=FACE_OUTER_BOUND ( 'NONE', #9733, .T. ) ;
#54991=CARTESIAN_POINT ( 'NONE',  ( -3.550000000000028688, 2.500000000000000000, 6.941600689897073018 ) ) ;
#54992=VERTEX_POINT ( 'NONE', #98692 ) ;
#54993=DIRECTION ( 'NONE',  ( -0.000000000000000000, 1.000000000000000000, -0.000000000000000000 ) ) ;
#54994=EDGE_CURVE ( 'NONE', #58972, #33187, #9688, .T. ) ;
#54995=DIRECTION ( 'NONE',  ( 0.000000000000000000, 0.000000000000000000, -1.000000000000000000 ) ) ;
#54996=AXIS2_PLACEMENT_3D ( 'NONE', #37818, #38489, #87551 ) ;
#54997=LINE ( 'NONE', #54354, #60444 ) ;
#54998=VERTEX_POINT ( 'NONE', #49633 ) ;
#54999=AXIS2_PLACEMENT_3D ( 'NONE', #68653, #128239, #58838 ) ;
#55000=AXIS2_PLACEMENT_3D ( 'NONE', #110480, #12268, #82966 ) ;
#55001=ORIENTED_EDGE ( 'NONE', *, *, #64487, .T. ) ;
#55002=ORIENTED_EDGE ( 'NONE', *, *, #17923, .F. ) ;
#55003=CARTESIAN_POINT ( 'NONE',  ( -2.499999999999996003, 2.500000000000000000, -4.330127018922201643 ) ) ;
#55004=CARTESIAN_POINT ( 'NONE',  ( 6.249999999999932498, 12.50000000000000000, -5.867463478539787225 ) ) ;
#55005=CARTESIAN_POINT ( 'NONE',  ( -4.600000000000024514, 2.500000000000000000, -0.7928203230275543412 ) ) ;
#55006=AXIS2_PLACEMENT_3D ( 'NONE', #27227, #76982, #30966 ) ;
#55007=ORIENTED_EDGE ( 'NONE', *, *, #59462, .T. ) ;
#55008=DIRECTION ( 'NONE',  ( 0.000000000000000000, 0.000000000000000000, -1.000000000000000000 ) ) ;
#55009=DIRECTION ( 'NONE',  ( -0.000000000000000000, -1.000000000000000000, -0.000000000000000000 ) ) ;
#55010=DIRECTION ( 'NONE',  ( 0.000000000000000000, 0.000000000000000000, 1.000000000000000000 ) ) ;
#55011=DIRECTION ( 'NONE',  ( 0.000000000000000000, 0.000000000000000000, 1.000000000000000000 ) ) ;
#55012=DIRECTION ( 'NONE',  ( 0.000000000000000000, 0.000000000000000000, 1.000000000000000000 ) ) ;
#55013=ADVANCED_FACE ( 'NONE', ( #18206 ), #96977, .T. ) ;
#55014=ORIENTED_EDGE ( 'NONE', *, *, #54307, .T. ) ;
#55015=DIRECTION ( 'NONE',  ( 0.000000000000000000, 0.000000000000000000, 1.000000000000000000 ) ) ;
#55016=ORIENTED_EDGE ( 'NONE', *, *, #61874, .F. ) ;
#55017=ORIENTED_EDGE ( 'NONE', *, *, #60662, .F. ) ;
#55018=ORIENTED_EDGE ( 'NONE', *, *, #102451, .T. ) ;
#55019=CONICAL_SURFACE ( 'NONE', #46718, 0.09999999999999982514, 0.003490658503988666988 ) ;
#55020=EDGE_CURVE ( 'NONE', #27555, #110342, #836, .T. ) ;
#55021=DIRECTION ( 'NONE',  ( 0.000000000000000000, 1.000000000000000000, 0.000000000000000000 ) ) ;
#55022=EDGE_CURVE ( 'NONE', #47693, #57040, #88214, .T. ) ;
#55023=FACE_BOUND ( 'NONE', #69312, .T. ) ;
#55024=ADVANCED_FACE ( 'NONE', ( #79716 ), #78118, .T. ) ;
#55025=DIRECTION ( 'NONE',  ( -4.274815082592931898E-19, -0.9999939076577903929, -0.003490651415223739937 ) ) ;
#55026=CARTESIAN_POINT ( 'NONE',  ( -5.600000000000020073, 2.500000000000000000, -0.2464101615137782308 ) ) ;
#55028=CONICAL_SURFACE ( 'NONE', #15301, 0.1000000000000000472, 0.003490658503988666988 ) ;
#55029=AXIS2_PLACEMENT_3D ( 'NONE', #74867, #28836, #117826 ) ;
#55031=EDGE_CURVE ( 'NONE', #26852, #108534, #66657, .T. ) ;
#55032=AXIS2_PLACEMENT_3D ( 'NONE', #95879, #6814, #114854 ) ;
#55033=EDGE_CURVE ( 'NONE', #86633, #42165, #55221, .T. ) ;
#55034=EDGE_LOOP ( 'NONE', ( #35873, #121960 ) ) ;
#55035=CARTESIAN_POINT ( 'NONE',  ( -0.8500000000000390576, 12.50000000000000000, -2.230156782645139391 ) ) ;
#55036=DIRECTION ( 'NONE',  ( -0.000000000000000000, 1.000000000000000000, -0.000000000000000000 ) ) ;
#55037=EDGE_CURVE ( 'NONE', #122432, #115626, #128403, .T. ) ;
#55038=CARTESIAN_POINT ( 'NONE',  ( 14.14999999999989555, 12.50000000000000000, 2.230156782645134950 ) ) ;
#55039=CARTESIAN_POINT ( 'NONE',  ( -7.900000000000014566, 2.500000000000000000, -0.7928203230275542301 ) ) ;
#55040=EDGE_LOOP ( 'NONE', ( #42943, #36800, #106329, #108032 ) ) ;
#55041=AXIS2_PLACEMENT_3D ( 'NONE', #46464, #4581, #94278 ) ;
#55042=CARTESIAN_POINT ( 'NONE',  ( 6.249999999999932498, 12.50000000000000000, 5.737276932171707422 ) ) ;
#55043=AXIS2_PLACEMENT_3D ( 'NONE', #50590, #98394, #99712 ) ;
#55044=CIRCLE ( 'NONE', #46639, 0.06509327318403745899 ) ;
#55045=EDGE_CURVE ( 'NONE', #25337, #5713, #26751, .T. ) ;
#55046=DIRECTION ( 'NONE',  ( 0.000000000000000000, 0.000000000000000000, 1.000000000000000000 ) ) ;
#55047=AXIS2_PLACEMENT_3D ( 'NONE', #25980, #26615, #74434 ) ;
#55048=ORIENTED_EDGE ( 'NONE', *, *, #69494, .T. ) ;
#55049=CIRCLE ( 'NONE', #117725, 0.06509327318403745899 ) ;
#55050=DIRECTION ( 'NONE',  ( 0.000000000000000000, 0.000000000000000000, 1.000000000000000000 ) ) ;
#55051=ADVANCED_FACE ( 'NONE', ( #19501 ), #9029, .T. ) ;
#55052=ORIENTED_EDGE ( 'NONE', *, *, #66318, .F. ) ;
#55053=FACE_BOUND ( 'NONE', #63937, .T. ) ;
#55054=EDGE_CURVE ( 'NONE', #88607, #95487, #68598, .T. ) ;
#55055=AXIS2_PLACEMENT_3D ( 'NONE', #106193, #17789, #55795 ) ;
#55056=CARTESIAN_POINT ( 'NONE',  ( 6.649999999999928413, 2.500000000000000000, 1.472243186433545459 ) ) ;
#55057=VERTEX_POINT ( 'NONE', #18853 ) ;
#55058=PLANE ( 'NONE',  #56848 ) ;
#55059=CARTESIAN_POINT ( 'NONE',  ( 0.8499999999999527933, 12.50000000000000000, 7.253104124594885960 ) ) ;
#55060=VERTEX_POINT ( 'NONE', #117679 ) ;
#55061=EDGE_LOOP ( 'NONE', ( #102654, #109131 ) ) ;
#55063=AXIS2_PLACEMENT_3D ( 'NONE', #95126, #117296, #66926 ) ;
#55064=EDGE_LOOP ( 'NONE', ( #49775, #49942 ) ) ;
#55065=DIRECTION ( 'NONE',  ( 0.000000000000000000, 1.000000000000000000, 0.000000000000000000 ) ) ;
#55066=FACE_OUTER_BOUND ( 'NONE', #39946, .T. ) ;
#55067=DIRECTION ( 'NONE',  ( -0.000000000000000000, -1.000000000000000000, -0.000000000000000000 ) ) ;
#55068=PLANE ( 'NONE',  #21829 ) ;
#55069=DIRECTION ( 'NONE',  ( 0.000000000000000000, 1.000000000000000000, 0.000000000000000000 ) ) ;
#55071=CIRCLE ( 'NONE', #2841, 0.09999999999999999167 ) ;
#55072=VECTOR ( 'NONE', #19818, 1000.000000000000000 ) ;
#55073=VECTOR ( 'NONE', #108947, 1000.000000000000000 ) ;
#55074=VERTEX_POINT ( 'NONE', #29344 ) ;
#55075=ORIENTED_EDGE ( 'NONE', *, *, #86177, .F. ) ;
#55076=DIRECTION ( 'NONE',  ( -0.000000000000000000, -1.000000000000000000, -0.000000000000000000 ) ) ;
#55077=DIRECTION ( 'NONE',  ( 0.000000000000000000, -0.000000000000000000, 1.000000000000000000 ) ) ;
#55078=DIRECTION ( 'NONE',  ( 0.000000000000000000, 1.000000000000000000, 0.000000000000000000 ) ) ;
#55079=CARTESIAN_POINT ( 'NONE',  ( -10.40000000000000391, 2.500000000000000000, -3.537306695894645969 ) ) ;
#55080=ORIENTED_EDGE ( 'NONE', *, *, #67559, .F. ) ;
#55081=ORIENTED_EDGE ( 'NONE', *, *, #83503, .F. ) ;
#55082=FACE_BOUND ( 'NONE', #121450, .T. ) ;
#55083=EDGE_LOOP ( 'NONE', ( #111847, #51320 ) ) ;
#55084=CIRCLE ( 'NONE', #46675, 0.06509327318403745899 ) ;
#55085=LINE ( 'NONE', #46537, #47136 ) ;
#55087=CIRCLE ( 'NONE', #75915, 0.06509327318403745899 ) ;
#55088=ORIENTED_EDGE ( 'NONE', *, *, #51523, .F. ) ;
#55089=AXIS2_PLACEMENT_3D ( 'NONE', #110628, #28862, #20961 ) ;
#55090=DIRECTION ( 'NONE',  ( 0.000000000000000000, -0.9999939076577903929, 0.003490651415223739937 ) ) ;
#55091=DIRECTION ( 'NONE',  ( 0.000000000000000000, 1.000000000000000000, 0.000000000000000000 ) ) ;
#55092=EDGE_CURVE ( 'NONE', #64400, #31027, #13436, .T. ) ;
#55094=DIRECTION ( 'NONE',  ( 0.000000000000000000, 0.000000000000000000, 1.000000000000000000 ) ) ;
#55095=FACE_OUTER_BOUND ( 'NONE', #13176, .T. ) ;
#55096=EDGE_CURVE ( 'NONE', #104138, #9737, #32258, .T. ) ;
#55097=CARTESIAN_POINT ( 'NONE',  ( -3.350000000000028511, 2.500000000000000000, -2.857883832488653741 ) ) ;
#55099=CARTESIAN_POINT ( 'NONE',  ( -5.400000000000023448, 12.50000000000000000, -4.330127018922201643 ) ) ;
#55100=CIRCLE ( 'NONE', #97146, 0.1000000000000002554 ) ;
#55101=DIRECTION ( 'NONE',  ( 0.000000000000000000, -0.000000000000000000, 1.000000000000000000 ) ) ;
#55102=ORIENTED_EDGE ( 'NONE', *, *, #90846, .F. ) ;
#55103=ORIENTED_EDGE ( 'NONE', *, *, #114606, .T. ) ;
#55104=CARTESIAN_POINT ( 'NONE',  ( -8.950000000000006395, 2.500000000000000000, 6.841600689897072485 ) ) ;
#55105=CIRCLE ( 'NONE', #115630, 0.06509327318403745899 ) ;
#55106=ORIENTED_EDGE ( 'NONE', *, *, #108527, .T. ) ;
#55107=AXIS2_PLACEMENT_3D ( 'NONE', #36957, #115484, #124033 ) ;
#55108=AXIS2_PLACEMENT_3D ( 'NONE', #105165, #94066, #55432 ) ;
#55109=DIRECTION ( 'NONE',  ( 0.000000000000000000, -0.9999939076577903929, 0.003490651415223739937 ) ) ;
#55110=VERTEX_POINT ( 'NONE', #7742 ) ;
#55111=ORIENTED_EDGE ( 'NONE', *, *, #10716, .F. ) ;
#55112=ORIENTED_EDGE ( 'NONE', *, *, #57091, .T. ) ;
#55113=AXIS2_PLACEMENT_3D ( 'NONE', #118171, #88716, #18030 ) ;
#55114=CARTESIAN_POINT ( 'NONE',  ( -15.39999999999997904, 2.500000000000000000, -0.6928203230275519209 ) ) ;
#55115=CIRCLE ( 'NONE', #32146, 0.06509327318403745899 ) ;
#55116=CARTESIAN_POINT ( 'NONE',  ( -12.49999999999999289, 2.500000000000000000, 3.637306695894644726 ) ) ;
#55119=DIRECTION ( 'NONE',  ( 0.000000000000000000, 0.000000000000000000, 1.000000000000000000 ) ) ;
#55120=VERTEX_POINT ( 'NONE', #47689 ) ;
#55121=CARTESIAN_POINT ( 'NONE',  ( -5.400000000000023448, 2.500000000000000000, -4.330127018922201643 ) ) ;
#55122=ORIENTED_EDGE ( 'NONE', *, *, #88516, .T. ) ;
#55123=VERTEX_POINT ( 'NONE', #87589 ) ;
#55124=ORIENTED_EDGE ( 'NONE', *, *, #57985, .T. ) ;
#55125=CARTESIAN_POINT ( 'NONE',  ( -9.600000000000006750, 2.500000000000000000, -0.5928203230275542746 ) ) ;
#55126=AXIS2_PLACEMENT_3D ( 'NONE', #88937, #30029, #128888 ) ;
#55127=VECTOR ( 'NONE', #43836, 1000.000000000000000 ) ;
#55128=EDGE_LOOP ( 'NONE', ( #26975, #85874, #6380, #104310 ) ) ;
#55129=VERTEX_POINT ( 'NONE', #28044 ) ;
#55130=ORIENTED_EDGE ( 'NONE', *, *, #81842, .F. ) ;
#55131=EDGE_CURVE ( 'NONE', #65795, #124333, #99369, .T. ) ;
#55132=VECTOR ( 'NONE', #21884, 1000.000000000000000 ) ;
#55133=DIRECTION ( 'NONE',  ( -0.000000000000000000, 1.000000000000000000, -0.000000000000000000 ) ) ;
#55134=DIRECTION ( 'NONE',  ( -0.000000000000000000, -1.000000000000000000, -0.000000000000000000 ) ) ;
#55135=AXIS2_PLACEMENT_3D ( 'NONE', #74545, #35909, #126877 ) ;
#55136=CARTESIAN_POINT ( 'NONE',  ( -3.150000000000029221, 2.500000000000000000, 2.511473670974873507 ) ) ;
#55137=DIRECTION ( 'NONE',  ( 0.000000000000000000, 0.000000000000000000, -1.000000000000000000 ) ) ;
#55138=AXIS2_PLACEMENT_3D ( 'NONE', #56056, #63963, #35790 ) ;
#55139=CIRCLE ( 'NONE', #109420, 0.1000000000000000472 ) ;
#55140=FACE_OUTER_BOUND ( 'NONE', #24445, .T. ) ;
#55141=EDGE_LOOP ( 'NONE', ( #6160, #55915 ) ) ;
#55142=CARTESIAN_POINT ( 'NONE',  ( 5.849999999999935696, 12.50000000000000000, -6.430097255199264339 ) ) ;
#55143=EDGE_CURVE ( 'NONE', #26619, #93332, #59444, .T. ) ;
#55144=AXIS2_PLACEMENT_3D ( 'NONE', #7183, #18300, #27460 ) ;
#55145=AXIS2_PLACEMENT_3D ( 'NONE', #74117, #23077, #92450 ) ;
#55146=ORIENTED_EDGE ( 'NONE', *, *, #12456, .T. ) ;
#55147=DIRECTION ( 'NONE',  ( 0.000000000000000000, 0.000000000000000000, 1.000000000000000000 ) ) ;
#55148=CIRCLE ( 'NONE', #107365, 0.06509327318403745899 ) ;
#55149=ORIENTED_EDGE ( 'NONE', *, *, #93254, .F. ) ;
#55150=DIRECTION ( 'NONE',  ( -0.000000000000000000, 1.000000000000000000, -0.000000000000000000 ) ) ;
#55151=ORIENTED_EDGE ( 'NONE', *, *, #60088, .F. ) ;
#55152=EDGE_CURVE ( 'NONE', #19955, #24096, #53174, .T. ) ;
#55153=EDGE_CURVE ( 'NONE', #59948, #124302, #69887, .T. ) ;
#55154=VERTEX_POINT ( 'NONE', #119627 ) ;
#55155=CARTESIAN_POINT ( 'NONE',  ( 12.29999999999990123, 2.500000000000000000, 0.4464101615137735513 ) ) ;
#55156=CARTESIAN_POINT ( 'NONE',  ( 8.099999999999923261, 2.500000000000000000, -4.083716857408426826 ) ) ;
#55157=ADVANCED_FACE ( 'NONE', ( #2422 ), #17641, .T. ) ;
#55158=CARTESIAN_POINT ( 'NONE',  ( 9.999999999999916511, 12.50000000000000000, -0.7579135962115916003 ) ) ;
#55159=CARTESIAN_POINT ( 'NONE',  ( -4.400000000000025224, 2.500000000000000000, -0.2464101615137783419 ) ) ;
#55160=ORIENTED_EDGE ( 'NONE', *, *, #110458, .F. ) ;
#55162=CARTESIAN_POINT ( 'NONE',  ( 12.29999999999990123, 2.500000000000000000, 0.3464101615137735735 ) ) ;
#55163=PLANE ( 'NONE',  #22257 ) ;
#55164=ADVANCED_FACE ( 'NONE', ( #21436 ), #120063, .T. ) ;
#55165=CARTESIAN_POINT ( 'NONE',  ( -3.150000000000029221, 2.500000000000000000, -1.818653347947326138 ) ) ;
#55166=DIRECTION ( 'NONE',  ( 0.000000000000000000, -0.000000000000000000, 1.000000000000000000 ) ) ;
#55167=VECTOR ( 'NONE', #13157, 1000.000000000000000 ) ;
#55168=CARTESIAN_POINT ( 'NONE',  ( -10.40000000000000213, 12.50000000000000000, 4.330127018922196314 ) ) ;
#55169=VERTEX_POINT ( 'NONE', #42380 ) ;
#55170=ORIENTED_EDGE ( 'NONE', *, *, #102178, .F. ) ;
#55171=CIRCLE ( 'NONE', #21426, 0.06509327318403745899 ) ;
#55172=EDGE_LOOP ( 'NONE', ( #101242, #76948 ) ) ;
#55173=FACE_OUTER_BOUND ( 'NONE', #62640, .T. ) ;
#55174=CARTESIAN_POINT ( 'NONE',  ( -1.450000000000036371, 2.500000000000000000, 2.611473670974873151 ) ) ;
#55175=AXIS2_PLACEMENT_3D ( 'NONE', #2704, #32844, #123763 ) ;
#55177=CARTESIAN_POINT ( 'NONE',  ( -9.800000000000006040, 2.500000000000000000, 0.3464101615137735735 ) ) ;
#55178=DIRECTION ( 'NONE',  ( -0.000000000000000000, 1.000000000000000000, -0.000000000000000000 ) ) ;
#55179=CARTESIAN_POINT ( 'NONE',  ( -3.100000000000028955, 2.500000000000000000, 4.676537180435972552 ) ) ;
#55180=AXIS2_PLACEMENT_3D ( 'NONE', #58123, #108490, #28008 ) ;
#55181=LINE ( 'NONE', #57105, #80991 ) ;
#55182=ORIENTED_EDGE ( 'NONE', *, *, #68646, .F. ) ;
#55183=CONICAL_SURFACE ( 'NONE', #2956, 0.1000000000000000472, 0.003490658503988666988 ) ;
#55184=CONICAL_SURFACE ( 'NONE', #103205, 0.1000000000000002554, 0.003490658503988666988 ) ;
#55185=EDGE_CURVE ( 'NONE', #128715, #88410, #126325, .T. ) ;
#55186=DIRECTION ( 'NONE',  ( 0.000000000000000000, 0.000000000000000000, 1.000000000000000000 ) ) ;
#55187=CARTESIAN_POINT ( 'NONE',  ( -4.150000000000025224, 12.50000000000000000, 7.188010851410848723 ) ) ;
#55188=ORIENTED_EDGE ( 'NONE', *, *, #29183, .F. ) ;
#55189=EDGE_CURVE ( 'NONE', #65093, #115124, #76145, .T. ) ;
#55190=CARTESIAN_POINT ( 'NONE',  ( -2.050000000000032685, 2.500000000000000000, -6.595190528383302109 ) ) ;
#55192=EDGE_CURVE ( 'NONE', #90854, #108142, #122126, .T. ) ;
#55194=VERTEX_POINT ( 'NONE', #51561 ) ;
#55195=VECTOR ( 'NONE', #44088, 1000.000000000000000 ) ;
#55196=CIRCLE ( 'NONE', #32229, 0.06509327318403745899 ) ;
#55197=AXIS2_PLACEMENT_3D ( 'NONE', #110951, #59976, #80883 ) ;
#55198=DIRECTION ( 'NONE',  ( 0.000000000000000000, 0.000000000000000000, 1.000000000000000000 ) ) ;
#55199=ADVANCED_FACE ( 'NONE', ( #120926 ), #51122, .T. ) ;
#55200=ADVANCED_FACE ( 'NONE', ( #1155 ), #21781, .T. ) ;
#55201=VECTOR ( 'NONE', #74233, 1000.000000000000000 ) ;
#55202=ORIENTED_EDGE ( 'NONE', *, *, #126707, .T. ) ;
#55203=CARTESIAN_POINT ( 'NONE',  ( -6.650000000000015454, 2.500000000000000000, 7.288010851410849256 ) ) ;
#55204=DIRECTION ( 'NONE',  ( 0.000000000000000000, 0.000000000000000000, 1.000000000000000000 ) ) ;
#55205=EDGE_CURVE ( 'NONE', #114757, #4060, #9249, .T. ) ;
#55206=CARTESIAN_POINT ( 'NONE',  ( -10.85000000000000142, 2.500000000000000000, -2.857883832488649745 ) ) ;
#55207=ADVANCED_FACE ( 'NONE', ( #100009 ), #44857, .T. ) ;
#55208=CIRCLE ( 'NONE', #57347, 0.06509327318403745899 ) ;
#55209=ORIENTED_EDGE ( 'NONE', *, *, #8376, .F. ) ;
#55210=DIRECTION ( 'NONE',  ( 0.000000000000000000, 0.000000000000000000, 1.000000000000000000 ) ) ;
#55212=DIRECTION ( 'NONE',  ( 0.000000000000000000, 0.000000000000000000, 1.000000000000000000 ) ) ;
#55213=VERTEX_POINT ( 'NONE', #91467 ) ;
#55214=ADVANCED_FACE ( 'NONE', ( #101941 ), #61493, .T. ) ;
#55215=CARTESIAN_POINT ( 'NONE',  ( 4.149999999999941735, 2.500000000000000000, -2.757883832488654097 ) ) ;
#55216=EDGE_LOOP ( 'NONE', ( #35134, #103063, #12324, #107233 ) ) ;
#55217=ORIENTED_EDGE ( 'NONE', *, *, #22094, .T. ) ;
#55218=DIRECTION ( 'NONE',  ( 0.000000000000000000, -0.000000000000000000, 1.000000000000000000 ) ) ;
#55219=DIRECTION ( 'NONE',  ( 0.000000000000000000, 0.000000000000000000, 1.000000000000000000 ) ) ;
#55220=VECTOR ( 'NONE', #33272, 1000.000000000000000 ) ;
#55221=CIRCLE ( 'NONE', #44759, 0.06509327318403745899 ) ;
#55222=ORIENTED_EDGE ( 'NONE', *, *, #127023, .F. ) ;
#55223=CARTESIAN_POINT ( 'NONE',  ( 8.149999999999920419, 12.50000000000000000, 6.906693963081109722 ) ) ;
#55224=DIRECTION ( 'NONE',  ( 0.000000000000000000, -0.000000000000000000, 1.000000000000000000 ) ) ;
#55225=ORIENTED_EDGE ( 'NONE', *, *, #7825, .T. ) ;
#55226=DIRECTION ( 'NONE',  ( 0.000000000000000000, 0.000000000000000000, -1.000000000000000000 ) ) ;
#55227=CIRCLE ( 'NONE', #128408, 0.06509327318403745899 ) ;
#55228=FACE_OUTER_BOUND ( 'NONE', #33075, .T. ) ;
#55229=AXIS2_PLACEMENT_3D ( 'NONE', #12652, #21199, #92514 ) ;
#55230=AXIS2_PLACEMENT_3D ( 'NONE', #129354, #97926, #69759 ) ;
#55231=CARTESIAN_POINT ( 'NONE',  ( 6.699999999999930012, 12.50000000000000000, -4.330127018922201643 ) ) ;
#55232=CARTESIAN_POINT ( 'NONE',  ( -6.050000000000022027, 12.50000000000000000, -1.753560074763288679 ) ) ;
#55233=DIRECTION ( 'NONE',  ( 0.000000000000000000, -0.9999939076577903929, 0.003490651415223739937 ) ) ;
#55234=DIRECTION ( 'NONE',  ( 0.000000000000000000, 1.000000000000000000, 0.000000000000000000 ) ) ;
#55235=AXIS2_PLACEMENT_3D ( 'NONE', #51493, #69831, #11545 ) ;
#55236=CIRCLE ( 'NONE', #111758, 0.1000000000000002554 ) ;
#55237=CONICAL_SURFACE ( 'NONE', #117917, 0.1000000000000002554, 0.003490658503988666988 ) ;
#55238=ORIENTED_EDGE ( 'NONE', *, *, #106417, .T. ) ;
#55239=EDGE_LOOP ( 'NONE', ( #105250, #18392, #70336, #75907 ) ) ;
#55240=VERTEX_POINT ( 'NONE', #1784 ) ;
#55241=EDGE_LOOP ( 'NONE', ( #28530, #50011, #71948, #22106 ) ) ;
#55242=PLANE ( 'NONE',  #95488 ) ;
#55243=CARTESIAN_POINT ( 'NONE',  ( -8.950000000000011724, 2.500000000000000000, -6.248780366869521430 ) ) ;
#55244=LINE ( 'NONE', #115406, #34285 ) ;
#55245=ORIENTED_EDGE ( 'NONE', *, *, #64808, .F. ) ;
#55246=FACE_BOUND ( 'NONE', #91449, .T. ) ;
#55247=FACE_OUTER_BOUND ( 'NONE', #46321, .T. ) ;
#55248=DIRECTION ( 'NONE',  ( 0.000000000000000000, 0.000000000000000000, 1.000000000000000000 ) ) ;
#55249=CARTESIAN_POINT ( 'NONE',  ( -1.250000000000037526, 2.500000000000000000, -5.802370205355749988 ) ) ;
#55250=EDGE_CURVE ( 'NONE', #32033, #120581, #81645, .T. ) ;
#55251=DIRECTION ( 'NONE',  ( -0.000000000000000000, -1.000000000000000000, -0.000000000000000000 ) ) ;
#55252=DIRECTION ( 'NONE',  ( 0.05223670945016245515, 0.9986347311133432214, 0.000000000000000000 ) ) ;
#55253=CARTESIAN_POINT ( 'NONE',  ( 9.149999999999916866, 12.50000000000000000, -1.472243186433550122 ) ) ;
#55254=DIRECTION ( 'NONE',  ( 0.000000000000000000, 0.000000000000000000, 1.000000000000000000 ) ) ;
#55255=DIRECTION ( 'NONE',  ( -0.000000000000000000, -1.000000000000000000, -0.000000000000000000 ) ) ;
#55256=DIRECTION ( 'NONE',  ( 0.000000000000000000, 0.000000000000000000, -1.000000000000000000 ) ) ;
#55257=CIRCLE ( 'NONE', #21818, 0.06509327318403745899 ) ;
#55258=CARTESIAN_POINT ( 'NONE',  ( 7.299999999999927880, 2.500000000000000000, 3.983716857408420964 ) ) ;
#55259=EDGE_CURVE ( 'NONE', #93988, #84759, #30194, .T. ) ;
#55260=ORIENTED_EDGE ( 'NONE', *, *, #37784, .T. ) ;
#55261=ORIENTED_EDGE ( 'NONE', *, *, #59530, .F. ) ;
#55262=ORIENTED_EDGE ( 'NONE', *, *, #4356, .F. ) ;
#55263=VERTEX_POINT ( 'NONE', #80377 ) ;
#55264=DIRECTION ( 'NONE',  ( 0.000000000000000000, 0.000000000000000000, 1.000000000000000000 ) ) ;
#55265=ORIENTED_EDGE ( 'NONE', *, *, #116326, .F. ) ;
#55266=DIRECTION ( 'NONE',  ( 0.000000000000000000, 0.000000000000000000, -1.000000000000000000 ) ) ;
#55267=ORIENTED_EDGE ( 'NONE', *, *, #14852, .F. ) ;
#55268=VERTEX_POINT ( 'NONE', #71180 ) ;
#55269=DIRECTION ( 'NONE',  ( 0.000000000000000000, 0.000000000000000000, 1.000000000000000000 ) ) ;
#55270=AXIS2_PLACEMENT_3D ( 'NONE', #3087, #92088, #93394 ) ;
#55271=AXIS2_PLACEMENT_3D ( 'NONE', #21566, #101417, #22227 ) ;
#55272=LINE ( 'NONE', #115447, #112425 ) ;
#55273=CARTESIAN_POINT ( 'NONE',  ( -2.950000000000029932, 12.50000000000000000, 2.165063509461097713 ) ) ;
#55274=DIRECTION ( 'NONE',  ( -0.000000000000000000, -1.000000000000000000, -0.000000000000000000 ) ) ;
#55275=CARTESIAN_POINT ( 'NONE',  ( 11.64999999999990443, 2.500000000000000000, -5.802370205355749988 ) ) ;
#55276=ORIENTED_EDGE ( 'NONE', *, *, #58072, .F. ) ;
#55277=ORIENTED_EDGE ( 'NONE', *, *, #64270, .T. ) ;
#55278=AXIS2_PLACEMENT_3D ( 'NONE', #101721, #39600, #40217 ) ;
#55279=EDGE_LOOP ( 'NONE', ( #8800, #41833 ) ) ;
#55280=CARTESIAN_POINT ( 'NONE',  ( 11.84999999999990372, 2.500000000000000000, 2.411473670974873862 ) ) ;
#55283=ORIENTED_EDGE ( 'NONE', *, *, #24547, .T. ) ;
#55285=FACE_OUTER_BOUND ( 'NONE', #104149, .T. ) ;
#55286=DIRECTION ( 'NONE',  ( 0.000000000000000000, 1.000000000000000000, 0.000000000000000000 ) ) ;
#55287=CIRCLE ( 'NONE', #128462, 0.06509327318403745899 ) ;
#55288=DIRECTION ( 'NONE',  ( 0.000000000000000000, 0.000000000000000000, 1.000000000000000000 ) ) ;
#55289=AXIS2_PLACEMENT_3D ( 'NONE', #25944, #65851, #64562 ) ;
#55290=CARTESIAN_POINT ( 'NONE',  ( -0.4000000000000392131, 12.50000000000000000, -4.957854068765716882 ) ) ;
#55291=CARTESIAN_POINT ( 'NONE',  ( 1.849999999999948130, 12.50000000000000000, 6.148780366869520009 ) ) ;
#55292=CIRCLE ( 'NONE', #107514, 0.1000000000000002554 ) ;
#55293=ORIENTED_EDGE ( 'NONE', *, *, #53248, .F. ) ;
#55294=CIRCLE ( 'NONE', #28194, 0.06509327318403745899 ) ;
#55295=CARTESIAN_POINT ( 'NONE',  ( 6.849999999999930367, 2.500000000000000000, -6.941600689897078347 ) ) ;
#55296=ADVANCED_FACE ( 'NONE', ( #70537 ), #113806, .T. ) ;
#55297=ORIENTED_EDGE ( 'NONE', *, *, #34209, .T. ) ;
#55298=DIRECTION ( 'NONE',  ( 0.000000000000000000, -0.9999939076577903929, 0.003490651415223739937 ) ) ;
#55299=ORIENTED_EDGE ( 'NONE', *, *, #111522, .T. ) ;
#55301=DIRECTION ( 'NONE',  ( -0.000000000000000000, -1.000000000000000000, -0.000000000000000000 ) ) ;
#55302=ORIENTED_EDGE ( 'NONE', *, *, #73326, .T. ) ;
#55303=DIRECTION ( 'NONE',  ( 0.000000000000000000, 0.000000000000000000, 1.000000000000000000 ) ) ;
#55304=EDGE_CURVE ( 'NONE', #10784, #126618, #73749, .T. ) ;
#55305=DIRECTION ( 'NONE',  ( 0.000000000000000000, 0.000000000000000000, -1.000000000000000000 ) ) ;
#55306=EDGE_CURVE ( 'NONE', #112093, #56250, #80360, .T. ) ;
#55307=ORIENTED_EDGE ( 'NONE', *, *, #90621, .T. ) ;
#55308=CONICAL_SURFACE ( 'NONE', #63908, 0.1000000000000002554, 0.003490658503988666988 ) ;
#55309=EDGE_CURVE ( 'NONE', #123444, #124385, #3729, .T. ) ;
#55310=VECTOR ( 'NONE', #67857, 1000.000000000000000 ) ;
#55311=FACE_OUTER_BOUND ( 'NONE', #9931, .T. ) ;
#55312=ORIENTED_EDGE ( 'NONE', *, *, #87597, .T. ) ;
#55313=ORIENTED_EDGE ( 'NONE', *, *, #49920, .T. ) ;
#55314=VECTOR ( 'NONE', #114845, 1000.000000000000000 ) ;
#55315=CIRCLE ( 'NONE', #30285, 0.1000000000000002554 ) ;
#55316=ORIENTED_EDGE ( 'NONE', *, *, #38690, .T. ) ;
#55318=DIRECTION ( 'NONE',  ( 0.000000000000000000, 0.000000000000000000, -1.000000000000000000 ) ) ;
#55319=EDGE_CURVE ( 'NONE', #77958, #9996, #929, .T. ) ;
#55321=CARTESIAN_POINT ( 'NONE',  ( 10.39999999999991154, 2.500000000000000000, 5.022947341949748790 ) ) ;
#55322=CONICAL_SURFACE ( 'NONE', #80368, 0.1000000000000002554, 0.003490658503988666988 ) ;
#55323=DIRECTION ( 'NONE',  ( 0.000000000000000000, 1.000000000000000000, 0.000000000000000000 ) ) ;
#55324=CIRCLE ( 'NONE', #34694, 0.06509327318403745899 ) ;
#55325=AXIS2_PLACEMENT_3D ( 'NONE', #34911, #6054, #15883 ) ;
#55326=LINE ( 'NONE', #115503, #79991 ) ;
#55327=AXIS2_PLACEMENT_3D ( 'NONE', #128927, #16962, #116482 ) ;
#55328=ORIENTED_EDGE ( 'NONE', *, *, #48330, .T. ) ;
#55329=AXIS2_PLACEMENT_3D ( 'NONE', #120348, #81069, #91525 ) ;
#55330=CARTESIAN_POINT ( 'NONE',  ( -0.6000000000000388356, 2.500000000000000000, 4.083716857408421497 ) ) ;
#55331=VECTOR ( 'NONE', #13682, 1000.000000000000000 ) ;
#55332=ORIENTED_EDGE ( 'NONE', *, *, #68678, .T. ) ;
#55333=CIRCLE ( 'NONE', #61605, 0.09999999999999982514 ) ;
#55334=CARTESIAN_POINT ( 'NONE',  ( -2.300000000000033573, 2.500000000000000000, 4.576537180435972019 ) ) ;
#55336=LINE ( 'NONE', #35697, #100283 ) ;
#55337=VERTEX_POINT ( 'NONE', #83596 ) ;
#55338=DIRECTION ( 'NONE',  ( -0.000000000000000000, -1.000000000000000000, -0.000000000000000000 ) ) ;
#55339=CARTESIAN_POINT ( 'NONE',  ( -7.050000000000016698, 2.500000000000000000, -2.165063509461101710 ) ) ;
#55340=AXIS2_PLACEMENT_3D ( 'NONE', #76081, #45986, #16487 ) ;
#55341=EDGE_LOOP ( 'NONE', ( #104984, #104030, #76347, #4469 ) ) ;
#55342=DIRECTION ( 'NONE',  ( 0.000000000000000000, -0.000000000000000000, 1.000000000000000000 ) ) ;
#55343=EDGE_LOOP ( 'NONE', ( #92169, #66750 ) ) ;
#55344=EDGE_LOOP ( 'NONE', ( #93819, #111095, #125102, #35653 ) ) ;
#55345=LINE ( 'NONE', #104442, #50833 ) ;
#55346=EDGE_CURVE ( 'NONE', #81635, #92156, #74093, .T. ) ;
#55347=ADVANCED_FACE ( 'NONE', ( #5650 ), #25979, .T. ) ;
#55348=ORIENTED_EDGE ( 'NONE', *, *, #109686, .T. ) ;
#55349=CARTESIAN_POINT ( 'NONE',  ( 17.34645602450336810, 0.4686430837608600575, -5.377443133677279441 ) ) ;
#55351=ADVANCED_FACE ( 'NONE', ( #63950 ), #15581, .T. ) ;
#55352=DIRECTION ( 'NONE',  ( -0.000000000000000000, -1.000000000000000000, -0.000000000000000000 ) ) ;
#55353=CIRCLE ( 'NONE', #120203, 7.500000000000000000 ) ;
#55354=VERTEX_POINT ( 'NONE', #24670 ) ;
#55355=FACE_BOUND ( 'NONE', #119302, .T. ) ;
#55356=ADVANCED_FACE ( 'NONE', ( #44296 ), #101378, .T. ) ;
#55357=DIRECTION ( 'NONE',  ( 0.000000000000000000, 0.000000000000000000, -1.000000000000000000 ) ) ;
#55358=ORIENTED_EDGE ( 'NONE', *, *, #77091, .T. ) ;
#55359=CARTESIAN_POINT ( 'NONE',  ( 12.09999999999990195, 2.500000000000000000, 0.5928203230275495006 ) ) ;
#55360=DIRECTION ( 'NONE',  ( 0.000000000000000000, 0.000000000000000000, 1.000000000000000000 ) ) ;
#55361=ORIENTED_EDGE ( 'NONE', *, *, #103795, .T. ) ;
#55362=ADVANCED_FACE ( 'NONE', ( #122874 ), #88759, .T. ) ;
#55363=CIRCLE ( 'NONE', #7220, 0.06509327318403745899 ) ;
#55364=EDGE_CURVE ( 'NONE', #37337, #92847, #103875, .T. ) ;
#55365=VERTEX_POINT ( 'NONE', #33217 ) ;
#55366=AXIS2_PLACEMENT_3D ( 'NONE', #124301, #104016, #74549 ) ;
#55367=EDGE_LOOP ( 'NONE', ( #178, #8710, #86000, #109555 ) ) ;
#55368=FACE_OUTER_BOUND ( 'NONE', #118560, .T. ) ;
#55369=DIRECTION ( 'NONE',  ( -0.000000000000000000, 1.000000000000000000, -0.000000000000000000 ) ) ;
#55370=CARTESIAN_POINT ( 'NONE',  ( 7.499999999999961808, 12.50000000000000000, 4.330127018922196314 ) ) ;
#55371=FACE_BOUND ( 'NONE', #105215, .T. ) ;
#55372=ORIENTED_EDGE ( 'NONE', *, *, #99248, .T. ) ;
#55374=ADVANCED_FACE ( 'NONE', ( #115607 ), #125441, .T. ) ;
#55375=DIRECTION ( 'NONE',  ( 0.000000000000000000, 0.000000000000000000, 1.000000000000000000 ) ) ;
#55376=CARTESIAN_POINT ( 'NONE',  ( -8.350000000000010303, 2.500000000000000000, 6.495190528383297135 ) ) ;
#55377=CARTESIAN_POINT ( 'NONE',  ( -12.89999999999999325, 2.500000000000000000, 0.5928203230275536084 ) ) ;
#55378=AXIS2_PLACEMENT_3D ( 'NONE', #104467, #2545, #42517 ) ;
#55379=CONICAL_SURFACE ( 'NONE', #49137, 0.1000000000000002554, 0.003490658503988666988 ) ;
#55380=CARTESIAN_POINT ( 'NONE',  ( 4.349999999999938360, 2.500000000000000000, 1.718653347947321386 ) ) ;
#55381=CARTESIAN_POINT ( 'NONE',  ( -8.300000000000009592, 12.50000000000000000, 4.330127018922196314 ) ) ;
#55382=FACE_OUTER_BOUND ( 'NONE', #2925, .T. ) ;
#55383=CARTESIAN_POINT ( 'NONE',  ( 2.949999999999945111, 12.50000000000000000, 2.230156782645134950 ) ) ;
#55384=AXIS2_PLACEMENT_3D ( 'NONE', #50087, #955, #292 ) ;
#55385=CARTESIAN_POINT ( 'NONE',  ( 5.199999999999931788, 2.500000000000000000, 4.776537180435972196 ) ) ;
#55386=ORIENTED_EDGE ( 'NONE', *, *, #45128, .F. ) ;
#55387=ORIENTED_EDGE ( 'NONE', *, *, #7424, .T. ) ;
#55388=EDGE_LOOP ( 'NONE', ( #8360, #49520, #67590, #122372 ) ) ;
#55390=ORIENTED_EDGE ( 'NONE', *, *, #30393, .T. ) ;
#55392=CARTESIAN_POINT ( 'NONE',  ( 3.349999999999945466, 2.500000000000000000, -6.495190528383302464 ) ) ;
#55393=EDGE_LOOP ( 'NONE', ( #92172, #66396, #91955, #90737 ) ) ;
#55394=FACE_BOUND ( 'NONE', #101482, .T. ) ;
#55395=DIRECTION ( 'NONE',  ( 0.000000000000000000, 0.000000000000000000, 1.000000000000000000 ) ) ;
#55396=CIRCLE ( 'NONE', #34483, 0.1000000000000002554 ) ;
#55397=DIRECTION ( 'NONE',  ( 0.000000000000000000, 0.000000000000000000, 1.000000000000000000 ) ) ;
#55398=CIRCLE ( 'NONE', #116031, 0.09999999999999982514 ) ;
#55399=ORIENTED_EDGE ( 'NONE', *, *, #54265, .F. ) ;
#55400=AXIS2_PLACEMENT_3D ( 'NONE', #120462, #119173, #57687 ) ;
#55401=CARTESIAN_POINT ( 'NONE',  ( -6.850000000000017408, 2.500000000000000000, -2.411473670974877859 ) ) ;
#55402=DIRECTION ( 'NONE',  ( 0.000000000000000000, 0.000000000000000000, 1.000000000000000000 ) ) ;
#55403=FACE_OUTER_BOUND ( 'NONE', #69421, .T. ) ;
#55404=ORIENTED_EDGE ( 'NONE', *, *, #58573, .T. ) ;
#55405=DIRECTION ( 'NONE',  ( -0.000000000000000000, -1.000000000000000000, -0.000000000000000000 ) ) ;
#55406=AXIS2_PLACEMENT_3D ( 'NONE', #10670, #31013, #80742 ) ;
#55408=ADVANCED_FACE ( 'NONE', ( #94686 ), #65874, .T. ) ;
#55409=CIRCLE ( 'NONE', #5218, 0.06509327318403745899 ) ;
#55410=ORIENTED_EDGE ( 'NONE', *, *, #17003, .T. ) ;
#55411=ORIENTED_EDGE ( 'NONE', *, *, #42339, .F. ) ;
#55412=CARTESIAN_POINT ( 'NONE',  ( -1.850000000000033396, 2.500000000000000000, -6.941600689897077459 ) ) ;
#55413=AXIS2_PLACEMENT_3D ( 'NONE', #66590, #86873, #26676 ) ;
#55414=CARTESIAN_POINT ( 'NONE',  ( 1.249999999999988898, 2.500000000000000000, -6.395190528383301931 ) ) ;
#55415=CARTESIAN_POINT ( 'NONE',  ( -7.499999999999980460, 2.500000000000000000, 0.09999999999999772959 ) ) ;
#55416=EDGE_LOOP ( 'NONE', ( #105192, #124522 ) ) ;
#55417=CARTESIAN_POINT ( 'NONE',  ( 15.23091471424993060, 1.499999999999968026, -7.179421170830202925 ) ) ;
#55420=DIRECTION ( 'NONE',  ( 0.000000000000000000, -0.9999939076577903929, 0.003490651415223739937 ) ) ;
#55421=CARTESIAN_POINT ( 'NONE',  ( 2.899999999999945732, 2.500000000000000000, -4.330127018922201643 ) ) ;
#55423=DIRECTION ( 'NONE',  ( -0.000000000000000000, -1.000000000000000000, -0.000000000000000000 ) ) ;
#55425=CARTESIAN_POINT ( 'NONE',  ( -8.300000000000011369, 12.50000000000000000, -2.276824562219559311E-15 ) ) ;
#55426=ORIENTED_EDGE ( 'NONE', *, *, #108817, .T. ) ;
#55427=DIRECTION ( 'NONE',  ( 0.000000000000000000, 0.000000000000000000, 1.000000000000000000 ) ) ;
#55428=VERTEX_POINT ( 'NONE', #14811 ) ;
#55429=ORIENTED_EDGE ( 'NONE', *, *, #86352, .T. ) ;
#55430=DIRECTION ( 'NONE',  ( -0.000000000000000000, -1.000000000000000000, -0.000000000000000000 ) ) ;
#55431=DIRECTION ( 'NONE',  ( 0.000000000000000000, 0.000000000000000000, 1.000000000000000000 ) ) ;
#55432=DIRECTION ( 'NONE',  ( 0.000000000000000000, 0.000000000000000000, -1.000000000000000000 ) ) ;
#55433=DIRECTION ( 'NONE',  ( -0.000000000000000000, 1.000000000000000000, -0.000000000000000000 ) ) ;
#55434=ORIENTED_EDGE ( 'NONE', *, *, #104282, .F. ) ;
#55435=EDGE_LOOP ( 'NONE', ( #42854, #97130 ) ) ;
#55436=CARTESIAN_POINT ( 'NONE',  ( 0.6499999999999561684, 2.500000000000000000, -1.918653347947325782 ) ) ;
#55437=CARTESIAN_POINT ( 'NONE',  ( 65.38824919562647153, 3.824345297732404614, -5.305607913327973435 ) ) ;
#55438=LINE ( 'NONE', #4372, #87830 ) ;
#55439=VERTEX_POINT ( 'NONE', #82951 ) ;
#55440=EDGE_LOOP ( 'NONE', ( #45216, #29417, #104440, #116744 ) ) ;
#55441=CARTESIAN_POINT ( 'NONE',  ( 14.59999999999989484, 2.500000000000000000, 0.6928203230275494784 ) ) ;
#55442=CIRCLE ( 'NONE', #118226, 0.1000000000000002554 ) ;
#55443=CONICAL_SURFACE ( 'NONE', #105623, 0.1000000000000000472, 0.003490658503988666988 ) ;
#55444=VERTEX_POINT ( 'NONE', #54751 ) ;
#55445=DIRECTION ( 'NONE',  ( 0.000000000000000000, 0.000000000000000000, 1.000000000000000000 ) ) ;
#55446=CONICAL_SURFACE ( 'NONE', #34630, 0.1000000000000002554, 0.003490658503988666988 ) ;
#55447=EDGE_CURVE ( 'NONE', #14963, #72759, #35152, .T. ) ;
#55448=DIRECTION ( 'NONE',  ( -0.000000000000000000, -1.000000000000000000, -0.000000000000000000 ) ) ;
#55449=VERTEX_POINT ( 'NONE', #114960 ) ;
#55450=FACE_OUTER_BOUND ( 'NONE', #118997, .T. ) ;
#55451=DIRECTION ( 'NONE',  ( -0.000000000000000000, -1.000000000000000000, -0.000000000000000000 ) ) ;
#55452=CARTESIAN_POINT ( 'NONE',  ( -8.100000000000013856, 12.50000000000000000, -0.3464101615137782364 ) ) ;
#55453=ADVANCED_FACE ( 'NONE', ( #54125 ), #25286, .T. ) ;
#55454=PLANE ( 'NONE',  #75099 ) ;
#55455=EDGE_CURVE ( 'NONE', #26527, #93988, #53492, .T. ) ;
#55456=EDGE_LOOP ( 'NONE', ( #62490, #37567, #70692, #117843 ) ) ;
#55457=CIRCLE ( 'NONE', #126565, 0.06509327318403743123 ) ;
#55458=CARTESIAN_POINT ( 'NONE',  ( -12.89999999999999147, 2.500000000000000000, 3.537306695894645081 ) ) ;
#55459=CARTESIAN_POINT ( 'NONE',  ( -7.700000000000016165, 2.500000000000000000, 0.3464101615137735735 ) ) ;
#55460=AXIS2_PLACEMENT_3D ( 'NONE', #72629, #101438, #121709 ) ;
#55461=EDGE_CURVE ( 'NONE', #79663, #118275, #84647, .T. ) ;
#55462=ORIENTED_EDGE ( 'NONE', *, *, #3658, .F. ) ;
#55463=EDGE_CURVE ( 'NONE', #47559, #45160, #92972, .T. ) ;
#55464=ORIENTED_EDGE ( 'NONE', *, *, #34704, .T. ) ;
#55465=ADVANCED_FACE ( 'NONE', ( #128703 ), #99233, .T. ) ;
#55467=DIRECTION ( 'NONE',  ( 0.000000000000000000, 0.000000000000000000, -1.000000000000000000 ) ) ;
#55468=EDGE_CURVE ( 'NONE', #127925, #31177, #113900, .T. ) ;
#55469=DIRECTION ( 'NONE',  ( 0.000000000000000000, 0.000000000000000000, -1.000000000000000000 ) ) ;
#55470=EDGE_CURVE ( 'NONE', #59296, #70566, #8870, .T. ) ;
#55471=DIRECTION ( 'NONE',  ( -4.274815082592931898E-19, -0.9999939076577903929, -0.003490651415223739937 ) ) ;
#55472=CARTESIAN_POINT ( 'NONE',  ( -8.100000000000010303, 2.500000000000000000, 3.983716857408420964 ) ) ;
#55473=PLANE ( 'NONE',  #96615 ) ;
#55474=AXIS2_PLACEMENT_3D ( 'NONE', #37029, #76951, #27194 ) ;
#55475=AXIS2_PLACEMENT_3D ( 'NONE', #88560, #89850, #87267 ) ;
#55476=DIRECTION ( 'NONE',  ( 0.000000000000000000, -0.000000000000000000, 1.000000000000000000 ) ) ;
#55477=DIRECTION ( 'NONE',  ( 0.000000000000000000, 0.000000000000000000, 1.000000000000000000 ) ) ;
#55478=DIRECTION ( 'NONE',  ( 0.000000000000000000, -0.9999939076577903929, 0.003490651415223739937 ) ) ;
#55479=CARTESIAN_POINT ( 'NONE',  ( -11.89999999999999680, 2.500000000000000000, 0.4464101615137776591 ) ) ;
#55480=EDGE_CURVE ( 'NONE', #79987, #8533, #55315, .T. ) ;
#55481=CARTESIAN_POINT ( 'NONE',  ( -14.14999999999998614, 12.50000000000000000, 1.472243186433549456 ) ) ;
#55482=ORIENTED_EDGE ( 'NONE', *, *, #12471, .F. ) ;
#55483=CIRCLE ( 'NONE', #117270, 0.06509327318403745899 ) ;
#55484=ORIENTED_EDGE ( 'NONE', *, *, #25923, .F. ) ;
#55485=ORIENTED_EDGE ( 'NONE', *, *, #37727, .T. ) ;
#55486=DIRECTION ( 'NONE',  ( 0.000000000000000000, 1.000000000000000000, 0.000000000000000000 ) ) ;
#55487=CONICAL_SURFACE ( 'NONE', #3167, 0.09999999999999982514, 0.003490658503988666988 ) ;
#55489=ORIENTED_EDGE ( 'NONE', *, *, #22407, .F. ) ;
#55490=CARTESIAN_POINT ( 'NONE',  ( 12.04999999999990834, 2.500000000000000000, 6.395190528383296602 ) ) ;
#55491=CIRCLE ( 'NONE', #116027, 0.06509327318403745899 ) ;
#55492=AXIS2_PLACEMENT_3D ( 'NONE', #52576, #91221, #2836 ) ;
#55493=DIRECTION ( 'NONE',  ( -0.000000000000000000, -1.000000000000000000, -0.000000000000000000 ) ) ;
#55494=DIRECTION ( 'NONE',  ( 0.000000000000000000, 1.000000000000000000, 0.000000000000000000 ) ) ;
#55495=VERTEX_POINT ( 'NONE', #97908 ) ;
#55496=CARTESIAN_POINT ( 'NONE',  ( -1.850000000000033840, 2.500000000000000000, 6.148780366869520897 ) ) ;
#55497=ORIENTED_EDGE ( 'NONE', *, *, #110861, .T. ) ;
#55498=AXIS2_PLACEMENT_3D ( 'NONE', #5380, #23752, #25032 ) ;
#55499=AXIS2_PLACEMENT_3D ( 'NONE', #27380, #38541, #79097 ) ;
#55500=CIRCLE ( 'NONE', #128692, 0.06509327318403745899 ) ;
#55501=ORIENTED_EDGE ( 'NONE', *, *, #62715, .T. ) ;
#55503=EDGE_LOOP ( 'NONE', ( #54340, #89335, #104421, #100317 ) ) ;
#55504=CARTESIAN_POINT ( 'NONE',  ( 7.099999999999928590, 2.500000000000000000, -4.922947341949753586 ) ) ;
#55505=CIRCLE ( 'NONE', #5309, 0.06509327318403745899 ) ;
#55506=EDGE_CURVE ( 'NONE', #4351, #111323, #7263, .T. ) ;
#55507=CARTESIAN_POINT ( 'NONE',  ( 7.499999999999925393, 12.50000000000000000, 5.088040615133786027 ) ) ;
#55508=CARTESIAN_POINT ( 'NONE',  ( -1.050000000000038680, 12.50000000000000000, 6.776507416713035248 ) ) ;
#55509=EDGE_CURVE ( 'NONE', #20474, #68081, #38608, .T. ) ;
#55510=DIRECTION ( 'NONE',  ( -0.000000000000000000, 1.000000000000000000, -0.000000000000000000 ) ) ;
#55511=CIRCLE ( 'NONE', #95224, 7.500000000000000000 ) ;
#55512=VERTEX_POINT ( 'NONE', #36443 ) ;
#55513=EDGE_CURVE ( 'NONE', #114128, #120638, #19338, .T. ) ;
#55514=AXIS2_PLACEMENT_3D ( 'NONE', #4692, #124511, #44654 ) ;
#55515=CARTESIAN_POINT ( 'NONE',  ( -1.650000000000034328, 2.500000000000000000, -2.065063509461102065 ) ) ;
#55516=CONICAL_SURFACE ( 'NONE', #63923, 0.1000000000000002554, 0.003490658503988666988 ) ;
#55517=VERTEX_POINT ( 'NONE', #128020 ) ;
#55518=DIRECTION ( 'NONE',  ( 0.000000000000000000, 0.000000000000000000, 1.000000000000000000 ) ) ;
#55519=CARTESIAN_POINT ( 'NONE',  ( 15.23091471425135701, -1.500000000000127898, -7.179421170829354715 ) ) ;
#55520=FACE_OUTER_BOUND ( 'NONE', #8966, .T. ) ;
#55521=CARTESIAN_POINT ( 'NONE',  ( 15.05551045036142455, -2.483581587658090672, 4.666934263335505761 ) ) ;
#55522=EDGE_CURVE ( 'NONE', #7922, #111183, #76352, .T. ) ;
#55523=ADVANCED_FACE ( 'NONE', ( #47536 ), #80455, .T. ) ;
#55524=ORIENTED_EDGE ( 'NONE', *, *, #41174, .F. ) ;
#55525=EDGE_CURVE ( 'NONE', #50160, #6072, #120154, .T. ) ;
#55527=VERTEX_POINT ( 'NONE', #69090 ) ;
#55528=ORIENTED_EDGE ( 'NONE', *, *, #26388, .F. ) ;
#55529=CARTESIAN_POINT ( 'NONE',  ( -7.900000000000014566, 2.500000000000000000, -5.122947341949753763 ) ) ;
#55530=FACE_OUTER_BOUND ( 'NONE', #41991, .T. ) ;
#55531=LINE ( 'NONE', #45074, #27339 ) ;
#55532=FACE_BOUND ( 'NONE', #57665, .T. ) ;
#55533=DIRECTION ( 'NONE',  ( 0.000000000000000000, 0.000000000000000000, 1.000000000000000000 ) ) ;
#55534=VECTOR ( 'NONE', #70055, 1000.000000000000000 ) ;
#55535=CARTESIAN_POINT ( 'NONE',  ( -3.950000000000026379, 2.500000000000000000, 6.841600689897072485 ) ) ;
#55536=EDGE_CURVE ( 'NONE', #45787, #109690, #97165, .T. ) ;
#55537=DIRECTION ( 'NONE',  ( 0.000000000000000000, 1.000000000000000000, 0.000000000000000000 ) ) ;
#55538=CARTESIAN_POINT ( 'NONE',  ( -1.450000000000035483, 2.500000000000000000, 6.148780366869520897 ) ) ;
#55540=AXIS2_PLACEMENT_3D ( 'NONE', #19673, #90318, #30797 ) ;
#55541=CARTESIAN_POINT ( 'NONE',  ( -5.850000000000021849, 12.50000000000000000, -1.472243186433550122 ) ) ;
#55542=DIRECTION ( 'NONE',  ( -0.000000000000000000, -1.000000000000000000, -0.000000000000000000 ) ) ;
#55543=AXIS2_PLACEMENT_3D ( 'NONE', #27081, #4190, #64418 ) ;
#55544=CARTESIAN_POINT ( 'NONE',  ( 10.64999999999991331, 2.500000000000000000, 6.841600689897072485 ) ) ;
#55545=AXIS2_PLACEMENT_3D ( 'NONE', #109461, #40747, #20436 ) ;
#55546=ORIENTED_EDGE ( 'NONE', *, *, #8777, .F. ) ;
#55547=ORIENTED_EDGE ( 'NONE', *, *, #13194, .F. ) ;
#55548=EDGE_LOOP ( 'NONE', ( #84462, #20338 ) ) ;
#55549=VERTEX_POINT ( 'NONE', #107074 ) ;
#55550=DIRECTION ( 'NONE',  ( 0.000000000000000000, -0.9999939076577903929, 0.003490651415223739937 ) ) ;
#55551=EDGE_CURVE ( 'NONE', #97470, #46758, #61587, .T. ) ;
#55552=FACE_BOUND ( 'NONE', #109631, .T. ) ;
#55553=DIRECTION ( 'NONE',  ( 0.000000000000000000, 1.000000000000000000, 0.000000000000000000 ) ) ;
#55554=CIRCLE ( 'NONE', #109935, 0.09999999999999999167 ) ;
#55555=CIRCLE ( 'NONE', #53408, 0.09999999999999982514 ) ;
#55556=ORIENTED_EDGE ( 'NONE', *, *, #15042, .T. ) ;
#55557=DIRECTION ( 'NONE',  ( 0.000000000000000000, 0.000000000000000000, 1.000000000000000000 ) ) ;
#55558=DIRECTION ( 'NONE',  ( 0.000000000000000000, 0.000000000000000000, 1.000000000000000000 ) ) ;
#55559=ORIENTED_EDGE ( 'NONE', *, *, #11487, .F. ) ;
#55561=FACE_OUTER_BOUND ( 'NONE', #7167, .T. ) ;
#55562=CIRCLE ( 'NONE', #57623, 0.06509327318403745899 ) ;
#55563=AXIS2_PLACEMENT_3D ( 'NONE', #45279, #43995, #24346 ) ;
#55564=ADVANCED_FACE ( 'NONE', ( #37076 ), #67913, .T. ) ;
#55565=ORIENTED_EDGE ( 'NONE', *, *, #60978, .T. ) ;
#55566=CARTESIAN_POINT ( 'NONE',  ( 13.34999999999990017, 2.500000000000000000, 2.857883832488649301 ) ) ;
#55567=DIRECTION ( 'NONE',  ( 0.000000000000000000, -0.9999939076577903929, 0.003490651415223739937 ) ) ;
#55568=VERTEX_POINT ( 'NONE', #37713 ) ;
#55569=CARTESIAN_POINT ( 'NONE',  ( 4.149999999999938183, 2.500000000000000000, 2.165063509461097713 ) ) ;
#55570=DIRECTION ( 'NONE',  ( -0.000000000000000000, -1.000000000000000000, -0.000000000000000000 ) ) ;
#55571=LINE ( 'NONE', #7093, #66072 ) ;
#55573=EDGE_LOOP ( 'NONE', ( #67208, #64032 ) ) ;
#55574=ADVANCED_FACE ( 'NONE', ( #18704 ), #98536, .T. ) ;
#55576=ORIENTED_EDGE ( 'NONE', *, *, #61293, .F. ) ;
#55577=DIRECTION ( 'NONE',  ( 0.000000000000000000, 0.000000000000000000, 1.000000000000000000 ) ) ;
#55578=CARTESIAN_POINT ( 'NONE',  ( -3.750000000000027534, 2.500000000000000000, 2.857883832488649301 ) ) ;
#55579=AXIS2_PLACEMENT_3D ( 'NONE', #122694, #94514, #44792 ) ;
#55580=VERTEX_POINT ( 'NONE', #88743 ) ;
#55581=VECTOR ( 'NONE', #64964, 1000.000000000000000 ) ;
#55583=DIRECTION ( 'NONE',  ( 0.000000000000000000, 0.000000000000000000, 1.000000000000000000 ) ) ;
#55584=DIRECTION ( 'NONE',  ( 0.000000000000000000, 0.000000000000000000, 1.000000000000000000 ) ) ;
#55585=CARTESIAN_POINT ( 'NONE',  ( 8.949999999999917577, 2.500000000000000000, 6.148780366869520009 ) ) ;
#55586=DIRECTION ( 'NONE',  ( -4.274815082592931898E-19, -0.9999939076577903929, -0.003490651415223739937 ) ) ;
#55587=FACE_OUTER_BOUND ( 'NONE', #114258, .T. ) ;
#55588=EDGE_LOOP ( 'NONE', ( #123425, #90404, #42534, #5139 ) ) ;
#55589=EDGE_LOOP ( 'NONE', ( #14290, #74837 ) ) ;
#55590=DIRECTION ( 'NONE',  ( -4.274815082592931898E-19, -0.9999939076577903929, -0.003490651415223739937 ) ) ;
#55591=DIRECTION ( 'NONE',  ( -0.000000000000000000, 1.000000000000000000, -0.000000000000000000 ) ) ;
#55592=DIRECTION ( 'NONE',  ( 0.000000000000000000, 0.000000000000000000, 1.000000000000000000 ) ) ;
#55593=EDGE_LOOP ( 'NONE', ( #6341, #97199, #108709, #16990 ) ) ;
#55594=VERTEX_POINT ( 'NONE', #49484 ) ;
#55595=ORIENTED_EDGE ( 'NONE', *, *, #65269, .F. ) ;
#55596=CARTESIAN_POINT ( 'NONE',  ( -6.850000000000017408, 12.50000000000000000, -2.576566944158915184 ) ) ;
#55597=AXIS2_PLACEMENT_3D ( 'NONE', #29715, #31035, #12004 ) ;
#55598=CARTESIAN_POINT ( 'NONE',  ( 4.149999999999941735, 2.500000000000000000, -7.188010851410854052 ) ) ;
#55599=CARTESIAN_POINT ( 'NONE',  ( 2.699999999999946443, 2.500000000000000000, 0.4464101615137735513 ) ) ;
#55600=EDGE_CURVE ( 'NONE', #93321, #90179, #123208, .T. ) ;
#55602=CARTESIAN_POINT ( 'NONE',  ( -12.49999999999995914, 12.50000000000000000, 1.843143693225357538E-15 ) ) ;
#55603=DIRECTION ( 'NONE',  ( -0.000000000000000000, -1.000000000000000000, -0.000000000000000000 ) ) ;
#55604=AXIS2_PLACEMENT_3D ( 'NONE', #79170, #97502, #47766 ) ;
#55605=CARTESIAN_POINT ( 'NONE',  ( 11.44999999999991047, 12.50000000000000000, 6.213873640053558134 ) ) ;
#55606=DIRECTION ( 'NONE',  ( 0.000000000000000000, 1.000000000000000000, 0.000000000000000000 ) ) ;
#55607=CARTESIAN_POINT ( 'NONE',  ( -14.39999999999998614, 12.50000000000000000, -0.3464101615137760715 ) ) ;
#55608=ORIENTED_EDGE ( 'NONE', *, *, #68372, .F. ) ;
#55609=CARTESIAN_POINT ( 'NONE',  ( 7.499999999999961808, 2.500000000000000000, 4.330127018922196314 ) ) ;
#55610=ADVANCED_FACE ( 'NONE', ( #79573 ), #78313, .T. ) ;
#55611=ORIENTED_EDGE ( 'NONE', *, *, #10512, .T. ) ;
#55612=EDGE_CURVE ( 'NONE', #27445, #17419, #115945, .T. ) ;
#55613=ORIENTED_EDGE ( 'NONE', *, *, #26353, .T. ) ;
#55614=EDGE_CURVE ( 'NONE', #97372, #101017, #65760, .T. ) ;
#55615=CARTESIAN_POINT ( 'NONE',  ( 1.049999999999953637, 12.50000000000000000, -1.883746621131363597 ) ) ;
#55616=DIRECTION ( 'NONE',  ( 0.000000000000000000, 0.000000000000000000, -1.000000000000000000 ) ) ;
#55617=ADVANCED_FACE ( 'NONE', ( #32907 ), #9330, .T. ) ;
#55618=CARTESIAN_POINT ( 'NONE',  ( -17.50000000000000000, 2.500000000000000000, 10.00000000000000178 ) ) ;
#55619=CARTESIAN_POINT ( 'NONE',  ( 0.8499999999999536815, 2.500000000000000000, 6.595190528383296780 ) ) ;
#55620=DIRECTION ( 'NONE',  ( 0.000000000000000000, 1.000000000000000000, 0.000000000000000000 ) ) ;
#55621=DIRECTION ( 'NONE',  ( 0.000000000000000000, 0.000000000000000000, -1.000000000000000000 ) ) ;
#55622=FACE_OUTER_BOUND ( 'NONE', #51984, .T. ) ;
#55623=ORIENTED_EDGE ( 'NONE', *, *, #116344, .T. ) ;
#55625=AXIS2_PLACEMENT_3D ( 'NONE', #21442, #90162, #120931 ) ;
#55626=EDGE_CURVE ( 'NONE', #32790, #36953, #74184, .T. ) ;
#55627=CIRCLE ( 'NONE', #32671, 0.06509327318403743123 ) ;
#55628=CIRCLE ( 'NONE', #3307, 0.06509327318403745899 ) ;
#55629=LINE ( 'NONE', #105376, #123025 ) ;
#55630=ADVANCED_FACE ( 'NONE', ( #44007 ), #114029, .T. ) ;
#55631=ORIENTED_EDGE ( 'NONE', *, *, #50687, .F. ) ;
#55632=ADVANCED_FACE ( 'NONE', ( #23713 ), #69986, .T. ) ;
#55633=ORIENTED_EDGE ( 'NONE', *, *, #4470, .F. ) ;
#55634=CIRCLE ( 'NONE', #76476, 0.06509327318403745899 ) ;
#55635=ORIENTED_EDGE ( 'NONE', *, *, #7734, .T. ) ;
#55636=ORIENTED_EDGE ( 'NONE', *, *, #41327, .F. ) ;
#55637=CARTESIAN_POINT ( 'NONE',  ( -8.950000000000004619, 12.50000000000000000, 6.083687093685483660 ) ) ;
#55638=DIRECTION ( 'NONE',  ( 0.000000000000000000, -0.000000000000000000, 1.000000000000000000 ) ) ;
#55640=CARTESIAN_POINT ( 'NONE',  ( 16.55874544816229488, 0.4845305829427787869, -6.091953208798931207 ) ) ;
#55641=CARTESIAN_POINT ( 'NONE',  ( 10.44999999999991402, 12.50000000000000000, 6.430097255199259010 ) ) ;
#55642=CIRCLE ( 'NONE', #93209, 0.06509327318403745899 ) ;
#55643=AXIS2_PLACEMENT_3D ( 'NONE', #128008, #50568, #106432 ) ;
#55644=DIRECTION ( 'NONE',  ( -0.000000000000000000, -1.000000000000000000, -0.000000000000000000 ) ) ;
#55645=VERTEX_POINT ( 'NONE', #82642 ) ;
#55646=DIRECTION ( 'NONE',  ( 0.000000000000000000, 1.000000000000000000, 0.000000000000000000 ) ) ;
#55647=DIRECTION ( 'NONE',  ( 0.000000000000000000, 0.000000000000000000, 1.000000000000000000 ) ) ;
#55648=DIRECTION ( 'NONE',  ( 0.000000000000000000, 1.000000000000000000, 0.000000000000000000 ) ) ;
#55649=ORIENTED_EDGE ( 'NONE', *, *, #37721, .F. ) ;
#55650=ORIENTED_EDGE ( 'NONE', *, *, #90793, .F. ) ;
#55651=ORIENTED_EDGE ( 'NONE', *, *, #106428, .T. ) ;
#55652=CARTESIAN_POINT ( 'NONE',  ( -11.24999999999996447, 12.50000000000000000, -2.099970236277060476 ) ) ;
#55653=CARTESIAN_POINT ( 'NONE',  ( 0.5999999999999551248, 2.500000000000000000, -4.676537180435978769 ) ) ;
#55654=CARTESIAN_POINT ( 'NONE',  ( 2.299999999999948752, 2.500000000000000000, 0.3464101615137735735 ) ) ;
#55655=VERTEX_POINT ( 'NONE', #39668 ) ;
#55656=DIRECTION ( 'NONE',  ( 0.000000000000000000, 0.000000000000000000, -1.000000000000000000 ) ) ;
#55657=DIRECTION ( 'NONE',  ( 0.000000000000000000, 0.000000000000000000, 1.000000000000000000 ) ) ;
#55659=DIRECTION ( 'NONE',  ( 0.000000000000000000, 0.000000000000000000, 1.000000000000000000 ) ) ;
#55660=CARTESIAN_POINT ( 'NONE',  ( 4.399999999999939071, 12.50000000000000000, 0.2813168883297362810 ) ) ;
#55662=ORIENTED_EDGE ( 'NONE', *, *, #7245, .F. ) ;
#55663=AXIS2_PLACEMENT_3D ( 'NONE', #95669, #105493, #93102 ) ;
#55664=CARTESIAN_POINT ( 'NONE',  ( -2.900000000000030553, 12.50000000000000000, 5.022947341949748790 ) ) ;
#55665=AXIS2_PLACEMENT_3D ( 'NONE', #110691, #111318, #51790 ) ;
#55666=EDGE_CURVE ( 'NONE', #118209, #43898, #78403, .T. ) ;
#55667=EDGE_LOOP ( 'NONE', ( #13169, #124339 ) ) ;
#55668=ORIENTED_EDGE ( 'NONE', *, *, #15535, .F. ) ;
#55669=VERTEX_POINT ( 'NONE', #13225 ) ;
#55670=DIRECTION ( 'NONE',  ( 0.000000000000000000, -0.9999939076577903929, 0.003490651415223739937 ) ) ;
#55671=FACE_BOUND ( 'NONE', #56012, .T. ) ;
#55672=LINE ( 'NONE', #75309, #113947 ) ;
#55673=FACE_OUTER_BOUND ( 'NONE', #105628, .T. ) ;
#55674=ADVANCED_FACE ( 'NONE', ( #109679 ), #93062, .T. ) ;
#55675=AXIS2_PLACEMENT_3D ( 'NONE', #79681, #20769, #91436 ) ;
#55676=CARTESIAN_POINT ( 'NONE',  ( -0.4000000000000331624, 2.500000000000000000, -0.7928203230275518987 ) ) ;
#55677=ORIENTED_EDGE ( 'NONE', *, *, #36007, .F. ) ;
#55678=DIRECTION ( 'NONE',  ( 0.000000000000000000, 1.000000000000000000, 0.000000000000000000 ) ) ;
#55679=CARTESIAN_POINT ( 'NONE',  ( 8.149999999999923972, 2.500000000000000000, -6.148780366869526226 ) ) ;
#55680=DIRECTION ( 'NONE',  ( 0.000000000000000000, -0.9999939076577903929, 0.003490651415223739937 ) ) ;
#55681=LINE ( 'NONE', #75962, #40620 ) ;
#55682=ORIENTED_EDGE ( 'NONE', *, *, #74556, .T. ) ;
#55683=AXIS2_PLACEMENT_3D ( 'NONE', #8605, #45994, #127761 ) ;
#55684=CIRCLE ( 'NONE', #15961, 0.06509327318403745899 ) ;
#55685=CARTESIAN_POINT ( 'NONE',  ( 6.449999999999931788, 12.50000000000000000, 6.083687093685482772 ) ) ;
#55686=VECTOR ( 'NONE', #16924, 1000.000000000000000 ) ;
#55687=CARTESIAN_POINT ( 'NONE',  ( -1.900000000000034994, 2.500000000000000000, -0.4464101615137783252 ) ) ;
#55688=ORIENTED_EDGE ( 'NONE', *, *, #104684, .F. ) ;
#55689=DIRECTION ( 'NONE',  ( 0.000000000000000000, 0.000000000000000000, 1.000000000000000000 ) ) ;
#55690=FACE_BOUND ( 'NONE', #36114, .T. ) ;
#55691=CARTESIAN_POINT ( 'NONE',  ( -11.64999999999999680, 2.500000000000000000, 2.065063509461097624 ) ) ;
#55692=ORIENTED_EDGE ( 'NONE', *, *, #82729, .F. ) ;
#55693=CARTESIAN_POINT ( 'NONE',  ( 3.149999999999946176, 2.500000000000000000, -1.818653347947325916 ) ) ;
#55694=CARTESIAN_POINT ( 'NONE',  ( -1.900000000000034994, 2.500000000000000000, -0.3464101615137783474 ) ) ;
#55695=ORIENTED_EDGE ( 'NONE', *, *, #68585, .F. ) ;
#55696=VERTEX_POINT ( 'NONE', #64272 ) ;
#55698=CIRCLE ( 'NONE', #66160, 0.06509327318403745899 ) ;
#55699=ORIENTED_EDGE ( 'NONE', *, *, #52657, .F. ) ;
#55701=CARTESIAN_POINT ( 'NONE',  ( 6.249999999999965361, 2.500000000000000000, 2.165063509461097713 ) ) ;
#55702=AXIS2_PLACEMENT_3D ( 'NONE', #38302, #97211, #67749 ) ;
#55703=EDGE_CURVE ( 'NONE', #54702, #54886, #11566, .T. ) ;
#55704=CARTESIAN_POINT ( 'NONE',  ( 13.34999999999989662, 2.500000000000000000, -2.857883832488653741 ) ) ;
#55705=DIRECTION ( 'NONE',  ( -0.000000000000000000, 1.000000000000000000, -0.000000000000000000 ) ) ;
#55706=CIRCLE ( 'NONE', #55625, 0.06509327318403745899 ) ;
#55707=DIRECTION ( 'NONE',  ( 0.000000000000000000, 1.000000000000000000, 0.000000000000000000 ) ) ;
#55708=CIRCLE ( 'NONE', #122624, 0.06509327318403745899 ) ;
#55709=CIRCLE ( 'NONE', #43136, 0.09999999999999982514 ) ;
#55711=CIRCLE ( 'NONE', #20222, 0.06509327318403741736 ) ;
#55712=VERTEX_POINT ( 'NONE', #3421 ) ;
#55713=DIRECTION ( 'NONE',  ( -0.000000000000000000, -1.000000000000000000, -0.000000000000000000 ) ) ;
#55714=DIRECTION ( 'NONE',  ( -0.000000000000000000, 1.000000000000000000, -0.000000000000000000 ) ) ;
#55715=PLANE ( 'NONE',  #120283 ) ;
#55716=ADVANCED_FACE ( 'NONE', ( #123825 ), #42908, .T. ) ;
#55717=CARTESIAN_POINT ( 'NONE',  ( 12.09999999999990195, 2.500000000000000000, 0.5928203230275495006 ) ) ;
#55718=ORIENTED_EDGE ( 'NONE', *, *, #51693, .F. ) ;
#55719=EDGE_LOOP ( 'NONE', ( #52756, #97601, #29994, #67356 ) ) ;
#55720=DIRECTION ( 'NONE',  ( 0.000000000000000000, -1.000000000000000000, 0.000000000000000000 ) ) ;
#55721=ORIENTED_EDGE ( 'NONE', *, *, #83190, .T. ) ;
#55722=EDGE_CURVE ( 'NONE', #60318, #16136, #57554, .T. ) ;
#55723=CARTESIAN_POINT ( 'NONE',  ( -6.900000000000015454, 2.500000000000000000, 3.983716857408420076 ) ) ;
#55724=DIRECTION ( 'NONE',  ( 0.000000000000000000, 1.000000000000000000, 0.000000000000000000 ) ) ;
#55725=AXIS2_PLACEMENT_3D ( 'NONE', #48614, #27657, #8025 ) ;
#55726=EDGE_LOOP ( 'NONE', ( #129448, #72611, #102667, #25656 ) ) ;
#55727=DIRECTION ( 'NONE',  ( -0.000000000000000000, -1.000000000000000000, -0.000000000000000000 ) ) ;
#55728=DIRECTION ( 'NONE',  ( 0.000000000000000000, -0.000000000000000000, 1.000000000000000000 ) ) ;
#55729=DIRECTION ( 'NONE',  ( 0.000000000000000000, 0.000000000000000000, 1.000000000000000000 ) ) ;
#55730=AXIS2_PLACEMENT_3D ( 'NONE', #28858, #30154, #108694 ) ;
#55731=CARTESIAN_POINT ( 'NONE',  ( -6.450000000000019718, 12.50000000000000000, -1.753560074763288679 ) ) ;
#55732=CARTESIAN_POINT ( 'NONE',  ( 6.649999999999930189, 2.500000000000000000, 5.702370205355745014 ) ) ;
#55733=LINE ( 'NONE', #85194, #89231 ) ;
#55734=EDGE_CURVE ( 'NONE', #60113, #88053, #84732, .T. ) ;
#55735=FACE_OUTER_BOUND ( 'NONE', #20182, .T. ) ;
#55736=CARTESIAN_POINT ( 'NONE',  ( 13.09999999999989839, 2.500000000000000000, 0.3464101615137735735 ) ) ;
#55737=DIRECTION ( 'NONE',  ( -0.000000000000000000, 1.000000000000000000, -0.000000000000000000 ) ) ;
#55738=VERTEX_POINT ( 'NONE', #73439 ) ;
#55739=VERTEX_POINT ( 'NONE', #24360 ) ;
#55740=CARTESIAN_POINT ( 'NONE',  ( 5.599999999999933031, 2.500000000000000000, -0.2464101615137783419 ) ) ;
#55741=ORIENTED_EDGE ( 'NONE', *, *, #123821, .F. ) ;
#55742=DIRECTION ( 'NONE',  ( 0.000000000000000000, 0.000000000000000000, -1.000000000000000000 ) ) ;
#55743=VERTEX_POINT ( 'NONE', #23069 ) ;
#55744=VERTEX_POINT ( 'NONE', #53185 ) ;
#55745=ORIENTED_EDGE ( 'NONE', *, *, #125123, .F. ) ;
#55747=FACE_OUTER_BOUND ( 'NONE', #115838, .T. ) ;
#55748=ADVANCED_FACE ( 'NONE', ( #43370 ), #83286, .T. ) ;
#55750=CARTESIAN_POINT ( 'NONE',  ( 1.649999999999951505, 12.50000000000000000, -2.857883832488653741 ) ) ;
#55751=CARTESIAN_POINT ( 'NONE',  ( -5.450000000000019718, 2.500000000000000000, 6.595190528383296780 ) ) ;
#55752=DIRECTION ( 'NONE',  ( -4.274815082592931898E-19, -0.9999939076577903929, -0.003490651415223739937 ) ) ;
#55753=ORIENTED_EDGE ( 'NONE', *, *, #64008, .T. ) ;
#55754=DIRECTION ( 'NONE',  ( -0.000000000000000000, 1.000000000000000000, -0.000000000000000000 ) ) ;
#55755=ORIENTED_EDGE ( 'NONE', *, *, #7632, .F. ) ;
#55756=EDGE_CURVE ( 'NONE', #18162, #40987, #122315, .T. ) ;
#55758=VERTEX_POINT ( 'NONE', #5980 ) ;
#55760=EDGE_LOOP ( 'NONE', ( #79442, #60893 ) ) ;
#55761=CARTESIAN_POINT ( 'NONE',  ( 3.749999999999942268, 12.50000000000000000, 1.407149913249508000 ) ) ;
#55762=EDGE_CURVE ( 'NONE', #68655, #88216, #36640, .T. ) ;
#55763=ORIENTED_EDGE ( 'NONE', *, *, #64490, .T. ) ;
#55764=EDGE_CURVE ( 'NONE', #39804, #78396, #13620, .T. ) ;
#55766=EDGE_CURVE ( 'NONE', #123894, #103956, #72129, .T. ) ;
#55767=EDGE_CURVE ( 'NONE', #45538, #9181, #14512, .T. ) ;
#55768=CARTESIAN_POINT ( 'NONE',  ( -3.750000000000025757, 2.500000000000000000, 1.472243186433545459 ) ) ;
#55769=CIRCLE ( 'NONE', #26524, 0.06509327318403745899 ) ;
#55770=VECTOR ( 'NONE', #14774, 1000.000000000000000 ) ;
#55771=CARTESIAN_POINT ( 'NONE',  ( 10.44999999999991047, 2.500000000000000000, 2.065063509461097624 ) ) ;
#55772=PLANE ( 'NONE',  #41704 ) ;
#55773=CARTESIAN_POINT ( 'NONE',  ( 0.3999999999999563904, 2.500000000000000000, 3.737306695894644371 ) ) ;
#55774=DIRECTION ( 'NONE',  ( 0.000000000000000000, 0.000000000000000000, -1.000000000000000000 ) ) ;
#55776=DIRECTION ( 'NONE',  ( 0.000000000000000000, 0.000000000000000000, 1.000000000000000000 ) ) ;
#55777=ORIENTED_EDGE ( 'NONE', *, *, #91982, .T. ) ;
#55778=EDGE_CURVE ( 'NONE', #51310, #44668, #45044, .T. ) ;
#55779=AXIS2_PLACEMENT_3D ( 'NONE', #55097, #125741, #14504 ) ;
#55780=CARTESIAN_POINT ( 'NONE',  ( -4.150000000000027889, 12.50000000000000000, -7.188010851410854052 ) ) ;
#55781=VECTOR ( 'NONE', #119871, 1000.000000000000000 ) ;
#55782=CIRCLE ( 'NONE', #82986, 0.06509327318403745899 ) ;
#55784=EDGE_LOOP ( 'NONE', ( #110309, #52985 ) ) ;
#55785=CARTESIAN_POINT ( 'NONE',  ( -12.09999999999999432, 12.50000000000000000, 4.957854068765711553 ) ) ;
#55786=AXIS2_PLACEMENT_3D ( 'NONE', #104332, #76168, #13367 ) ;
#55787=ADVANCED_FACE ( 'NONE', ( #114657 ), #25625, .T. ) ;
#55788=VERTEX_POINT ( 'NONE', #115954 ) ;
#55789=DIRECTION ( 'NONE',  ( 0.000000000000000000, 0.000000000000000000, -1.000000000000000000 ) ) ;
#55790=ORIENTED_EDGE ( 'NONE', *, *, #67555, .T. ) ;
#55791=EDGE_LOOP ( 'NONE', ( #61939, #116735 ) ) ;
#55792=EDGE_CURVE ( 'NONE', #78283, #77627, #40851, .T. ) ;
#55793=DIRECTION ( 'NONE',  ( 0.000000000000000000, 0.000000000000000000, -1.000000000000000000 ) ) ;
#55794=DIRECTION ( 'NONE',  ( 0.000000000000000000, -0.000000000000000000, -1.000000000000000000 ) ) ;
#55795=DIRECTION ( 'NONE',  ( 0.000000000000000000, 0.000000000000000000, -1.000000000000000000 ) ) ;
#55796=PLANE ( 'NONE',  #82236 ) ;
#55797=DIRECTION ( 'NONE',  ( 0.000000000000000000, -0.9999939076577903929, 0.003490651415223739937 ) ) ;
#55798=ORIENTED_EDGE ( 'NONE', *, *, #127941, .T. ) ;
#55799=DIRECTION ( 'NONE',  ( -0.000000000000000000, -1.000000000000000000, -0.000000000000000000 ) ) ;
#55800=DIRECTION ( 'NONE',  ( 0.000000000000000000, 1.000000000000000000, 0.000000000000000000 ) ) ;
#55801=DIRECTION ( 'NONE',  ( 0.000000000000000000, 0.000000000000000000, -1.000000000000000000 ) ) ;
#55802=CONICAL_SURFACE ( 'NONE', #5598, 0.1000000000000000472, 0.003490658503988666988 ) ;
#55803=CARTESIAN_POINT ( 'NONE',  ( 14.14999999999989200, 2.500000000000000000, -2.265063509461101798 ) ) ;
#55804=VECTOR ( 'NONE', #119808, 1000.000000000000000 ) ;
#55805=DIRECTION ( 'NONE',  ( -0.000000000000000000, 1.000000000000000000, -0.000000000000000000 ) ) ;
#55806=ORIENTED_EDGE ( 'NONE', *, *, #101290, .F. ) ;
#55807=CIRCLE ( 'NONE', #5606, 0.1000000000000000472 ) ;
#55808=ORIENTED_EDGE ( 'NONE', *, *, #95416, .T. ) ;
#55810=CIRCLE ( 'NONE', #66269, 0.09999999999999982514 ) ;
#55811=ORIENTED_EDGE ( 'NONE', *, *, #70059, .T. ) ;
#55812=AXIS2_PLACEMENT_3D ( 'NONE', #119618, #98682, #69223 ) ;
#55813=CARTESIAN_POINT ( 'NONE',  ( 0.6499999999999543920, 2.500000000000000000, 6.841600689897072485 ) ) ;
#55814=PLANE ( 'NONE',  #66869 ) ;
#55816=DIRECTION ( 'NONE',  ( 0.000000000000000000, 0.000000000000000000, -1.000000000000000000 ) ) ;
#55817=CONICAL_SURFACE ( 'NONE', #85060, 0.1000000000000002554, 0.003490658503988666988 ) ;
#55818=DIRECTION ( 'NONE',  ( -0.000000000000000000, -1.000000000000000000, -0.000000000000000000 ) ) ;
#55819=DIRECTION ( 'NONE',  ( 0.000000000000000000, 1.000000000000000000, 0.000000000000000000 ) ) ;
#55820=DIRECTION ( 'NONE',  ( -0.000000000000000000, -1.000000000000000000, -0.000000000000000000 ) ) ;
#55821=ORIENTED_EDGE ( 'NONE', *, *, #10270, .F. ) ;
#55822=AXIS2_PLACEMENT_3D ( 'NONE', #92387, #43953, #2719 ) ;
#55823=EDGE_CURVE ( 'NONE', #13248, #15249, #38706, .T. ) ;
#55824=CARTESIAN_POINT ( 'NONE',  ( -12.04999999999999538, 2.500000000000000000, 2.165063509461097713 ) ) ;
#55825=DIRECTION ( 'NONE',  ( 0.000000000000000000, 0.000000000000000000, 1.000000000000000000 ) ) ;
#55826=EDGE_CURVE ( 'NONE', #53805, #122392, #87128, .T. ) ;
#55827=ORIENTED_EDGE ( 'NONE', *, *, #104212, .T. ) ;
#55828=CARTESIAN_POINT ( 'NONE',  ( 9.599999999999914380, 12.50000000000000000, 3.637306695894644726 ) ) ;
#55829=DIRECTION ( 'NONE',  ( -0.000000000000000000, 1.000000000000000000, -0.000000000000000000 ) ) ;
#55830=CARTESIAN_POINT ( 'NONE',  ( 8.149999999999923972, 2.500000000000000000, 2.511473670974873507 ) ) ;
#55831=EDGE_LOOP ( 'NONE', ( #83075, #40668, #86925, #108827 ) ) ;
#55832=FACE_OUTER_BOUND ( 'NONE', #23168, .T. ) ;
#55833=ORIENTED_EDGE ( 'NONE', *, *, #111015, .T. ) ;
#55834=DIRECTION ( 'NONE',  ( 0.000000000000000000, 0.000000000000000000, -1.000000000000000000 ) ) ;
#55835=DIRECTION ( 'NONE',  ( 0.000000000000000000, 1.000000000000000000, 0.000000000000000000 ) ) ;
#55836=CONICAL_SURFACE ( 'NONE', #78848, 0.1000000000000002554, 0.003490658503988666988 ) ;
#55837=ORIENTED_EDGE ( 'NONE', *, *, #3778, .T. ) ;
#55838=DIRECTION ( 'NONE',  ( 0.000000000000000000, 0.000000000000000000, 1.000000000000000000 ) ) ;
#55839=CARTESIAN_POINT ( 'NONE',  ( -12.89999999999999147, 2.500000000000000000, 0.1000000000000018513 ) ) ;
#55840=EDGE_LOOP ( 'NONE', ( #20624, #18264, #97441, #52771 ) ) ;
#55841=VERTEX_POINT ( 'NONE', #4681 ) ;
#55842=CARTESIAN_POINT ( 'NONE',  ( 9.149999999999916866, 2.500000000000000000, -1.372243186433550033 ) ) ;
#55843=VECTOR ( 'NONE', #71198, 1000.000000000000000 ) ;
#55844=AXIS2_PLACEMENT_3D ( 'NONE', #113776, #84303, #24747 ) ;
#55845=VERTEX_POINT ( 'NONE', #117210 ) ;
#55846=DIRECTION ( 'NONE',  ( 0.000000000000000000, 1.000000000000000000, 0.000000000000000000 ) ) ;
#55847=DIRECTION ( 'NONE',  ( 0.000000000000000000, -0.9999939076577903929, 0.003490651415223739937 ) ) ;
#55848=ORIENTED_EDGE ( 'NONE', *, *, #63688, .F. ) ;
#55849=CARTESIAN_POINT ( 'NONE',  ( 4.149999999999939959, 12.50000000000000000, 2.857883832488649301 ) ) ;
#55850=DIRECTION ( 'NONE',  ( 0.000000000000000000, 0.000000000000000000, -1.000000000000000000 ) ) ;
#55851=ORIENTED_EDGE ( 'NONE', *, *, #62875, .F. ) ;
#55853=AXIS2_PLACEMENT_3D ( 'NONE', #111388, #62322, #112705 ) ;
#55854=FACE_OUTER_BOUND ( 'NONE', #17834, .T. ) ;
#55855=EDGE_CURVE ( 'NONE', #64926, #114462, #64908, .T. ) ;
#55856=CARTESIAN_POINT ( 'NONE',  ( 1.449999999999950440, 2.500000000000000000, 6.048780366869520364 ) ) ;
#55857=PLANE ( 'NONE',  #120384 ) ;
#55858=DIRECTION ( 'NONE',  ( 0.000000000000000000, 0.000000000000000000, 1.000000000000000000 ) ) ;
#55859=DIRECTION ( 'NONE',  ( 0.000000000000000000, 0.000000000000000000, 1.000000000000000000 ) ) ;
#55860=DIRECTION ( 'NONE',  ( 0.000000000000000000, 1.000000000000000000, 0.000000000000000000 ) ) ;
#55861=CIRCLE ( 'NONE', #26536, 0.1000000000000000056 ) ;
#55862=AXIS2_PLACEMENT_3D ( 'NONE', #24792, #83079, #122994 ) ;
#55863=ORIENTED_EDGE ( 'NONE', *, *, #80122, .F. ) ;
#55864=VERTEX_POINT ( 'NONE', #6601 ) ;
#55865=VERTEX_POINT ( 'NONE', #94368 ) ;
#55866=EDGE_LOOP ( 'NONE', ( #81923, #124082 ) ) ;
#55867=CARTESIAN_POINT ( 'NONE',  ( -13.09999999999999076, 12.50000000000000000, 4.611443907251934426 ) ) ;
#55868=CARTESIAN_POINT ( 'NONE',  ( -0.8500000000000386136, 2.500000000000000000, 7.088010851410848190 ) ) ;
#55869=EDGE_CURVE ( 'NONE', #103647, #87563, #15665, .T. ) ;
#55870=DIRECTION ( 'NONE',  ( 0.000000000000000000, 0.000000000000000000, -1.000000000000000000 ) ) ;
#55871=VERTEX_POINT ( 'NONE', #15147 ) ;
#55872=FACE_BOUND ( 'NONE', #13207, .T. ) ;
#55873=EDGE_CURVE ( 'NONE', #92109, #93629, #126426, .T. ) ;
#55874=PLANE ( 'NONE',  #106468 ) ;
#55875=CARTESIAN_POINT ( 'NONE',  ( 7.899999999999924860, 2.500000000000000000, 4.922947341949748257 ) ) ;
#55876=DIRECTION ( 'NONE',  ( 0.000000000000000000, 0.000000000000000000, -1.000000000000000000 ) ) ;
#55877=VECTOR ( 'NONE', #104347, 1000.000000000000000 ) ;
#55878=FACE_OUTER_BOUND ( 'NONE', #81677, .T. ) ;
#55879=DIRECTION ( 'NONE',  ( 0.000000000000000000, -0.9999939076577903929, 0.003490651415223739937 ) ) ;
#55880=CARTESIAN_POINT ( 'NONE',  ( -3.350000000000028955, 12.50000000000000000, -2.165063509461101710 ) ) ;
#55881=CARTESIAN_POINT ( 'NONE',  ( -0.8500000000000382805, 2.500000000000000000, -5.902370205355750521 ) ) ;
#55882=CARTESIAN_POINT ( 'NONE',  ( -11.84999999999999609, 12.50000000000000000, 6.148780366869520897 ) ) ;
#55883=EDGE_CURVE ( 'NONE', #43992, #28400, #126507, .T. ) ;
#55884=DIRECTION ( 'NONE',  ( -0.000000000000000000, 1.000000000000000000, -0.000000000000000000 ) ) ;
#55885=CIRCLE ( 'NONE', #1592, 0.06509327318403745899 ) ;
#55886=DIRECTION ( 'NONE',  ( -0.000000000000000000, -1.000000000000000000, -0.000000000000000000 ) ) ;
#55887=ORIENTED_EDGE ( 'NONE', *, *, #77573, .T. ) ;
#55888=AXIS2_PLACEMENT_3D ( 'NONE', #119395, #118764, #107665 ) ;
#55889=VERTEX_POINT ( 'NONE', #65559 ) ;
#55890=ORIENTED_EDGE ( 'NONE', *, *, #74565, .T. ) ;
#55891=ORIENTED_EDGE ( 'NONE', *, *, #57838, .F. ) ;
#55892=CARTESIAN_POINT ( 'NONE',  ( -11.44999999999999929, 12.50000000000000000, -6.148780366869522673 ) ) ;
#55893=ORIENTED_EDGE ( 'NONE', *, *, #78944, .T. ) ;
#55894=CARTESIAN_POINT ( 'NONE',  ( -5.450000000000019718, 2.500000000000000000, 6.595190528383296780 ) ) ;
#55895=EDGE_LOOP ( 'NONE', ( #72516, #26091, #99105, #22381 ) ) ;
#55896=AXIS2_PLACEMENT_3D ( 'NONE', #10775, #98520, #8854 ) ;
#55897=EDGE_LOOP ( 'NONE', ( #23831, #1221 ) ) ;
#55898=CARTESIAN_POINT ( 'NONE',  ( 12.29999999999990123, 12.50000000000000000, 0.3464101615137735735 ) ) ;
#55899=CONICAL_SURFACE ( 'NONE', #122803, 0.1000000000000000472, 0.003490658503988666988 ) ;
#55900=CONICAL_SURFACE ( 'NONE', #112344, 0.1000000000000002554, 0.003490658503988666988 ) ;
#55902=DIRECTION ( 'NONE',  ( 0.000000000000000000, 0.000000000000000000, 1.000000000000000000 ) ) ;
#55903=FACE_OUTER_BOUND ( 'NONE', #61533, .T. ) ;
#55904=CARTESIAN_POINT ( 'NONE',  ( -1.450000000000035927, 12.50000000000000000, -6.213873640053564351 ) ) ;
#55905=CARTESIAN_POINT ( 'NONE',  ( -14.14999999999998614, 12.50000000000000000, -2.230156782645137170 ) ) ;
#55906=AXIS2_PLACEMENT_3D ( 'NONE', #77789, #18877, #129519 ) ;
#55907=VERTEX_POINT ( 'NONE', #95675 ) ;
#55908=EDGE_LOOP ( 'NONE', ( #70529, #82026, #24129, #125265 ) ) ;
#55909=EDGE_CURVE ( 'NONE', #113368, #104854, #82597, .T. ) ;
#55910=AXIS2_PLACEMENT_3D ( 'NONE', #116128, #114831, #16625 ) ;
#55911=EDGE_LOOP ( 'NONE', ( #104851, #979, #39321, #7611 ) ) ;
#55912=EDGE_LOOP ( 'NONE', ( #8760, #77299 ) ) ;
#55913=DIRECTION ( 'NONE',  ( 0.9974916312695811804, -0.05217691604167150332, -0.04783319955355572195 ) ) ;
#55914=( BOUNDED_SURFACE ( )  B_SPLINE_SURFACE ( 3, 2, ( 
 ( #49250, #9951, #100268 ),
 ( #51180, #79975, #108781 ),
 ( #121187, #128458, #20419 ),
 ( #89152, #49893, #60976 ),
 ( #31526, #98314, #38798 ),
 ( #60363, #119903, #89795 ),
 ( #10572, #88498, #39442 ),
 ( #110084, #119250, #50508 ),
 ( #90419, #91086, #80636 ),
 ( #110715, #70799, #120548 ),
 ( #9211, #108700, #28867 ),
 ( #98231, #70071, #88397 ) ),
 .UNSPECIFIED., .F., .F., .F. ) 
 B_SPLINE_SURFACE_WITH_KNOTS ( ( 4, 2, 2, 2, 2, 4 ),
 ( 3, 3 ),
 ( 0.02236387153718017232, 0.03065407938765537382, 0.03894428723813057880, 0.05552470293908098875, 0.07210511864003139870, 0.08868553434098180865 ),
 ( 0.000000000000000000, 1.000000000000000000 ),
 .UNSPECIFIED. ) 
 GEOMETRIC_REPRESENTATION_ITEM ( )  RATIONAL_B_SPLINE_SURFACE ( (
 ( 1.000000000000000000, 0.7318752858502177716, 1.000000000000000000),
 ( 1.000000000000000000, 0.7503381610177722871, 1.000000000000000000),
 ( 1.000000000000000000, 0.7702514485279070566, 1.000000000000000000),
 ( 1.000000000000000000, 0.8097395513079956864, 1.000000000000000000),
 ( 1.000000000000000000, 0.8293075644331776575, 1.000000000000000000),
 ( 1.000000000000000000, 0.8842435496613439971, 1.000000000000000000),
 ( 1.000000000000000000, 0.9156028214505685936, 1.000000000000000000),
 ( 1.000000000000000000, 0.9624374057520458381, 1.000000000000000000),
 ( 1.000000000000000000, 0.9780629942474001748, 1.000000000000000000),
 ( 1.000000000000000000, 0.9967432622277094811, 1.000000000000000000),
 ( 1.000000000000000000, 0.9999962847131013133, 1.000000000000000000),
 ( 1.000000000000000000, 1.000000000000000000, 1.000000000000000000) ) ) 
 REPRESENTATION_ITEM ( '' )  SURFACE ( )  );
#55915=ORIENTED_EDGE ( 'NONE', *, *, #23802, .F. ) ;
#55916=EDGE_CURVE ( 'NONE', #3681, #6598, #86779, .T. ) ;
#55917=ORIENTED_EDGE ( 'NONE', *, *, #60903, .F. ) ;
#55918=EDGE_CURVE ( 'NONE', #103499, #23121, #88846, .T. ) ;
#55919=DIRECTION ( 'NONE',  ( 0.000000000000000000, -0.000000000000000000, 1.000000000000000000 ) ) ;
#55920=DIRECTION ( 'NONE',  ( 0.000000000000000000, 0.000000000000000000, 1.000000000000000000 ) ) ;
#55921=FACE_OUTER_BOUND ( 'NONE', #92686, .T. ) ;
#55922=DIRECTION ( 'NONE',  ( 0.000000000000000000, 0.000000000000000000, 1.000000000000000000 ) ) ;
#55923=ADVANCED_FACE ( 'NONE', ( #59644 ), #7921, .T. ) ;
#55924=EDGE_CURVE ( 'NONE', #6869, #88265, #65853, .T. ) ;
#55925=CARTESIAN_POINT ( 'NONE',  ( 12.94999999999990337, 12.50000000000000000, 2.099970236277060032 ) ) ;
#55926=DIRECTION ( 'NONE',  ( 0.000000000000000000, 0.000000000000000000, 1.000000000000000000 ) ) ;
#55927=EDGE_CURVE ( 'NONE', #26594, #123378, #80544, .T. ) ;
#55928=VERTEX_POINT ( 'NONE', #49811 ) ;
#55929=DIRECTION ( 'NONE',  ( 0.000000000000000000, 0.000000000000000000, 1.000000000000000000 ) ) ;
#55930=ORIENTED_EDGE ( 'NONE', *, *, #35679, .F. ) ;
#55931=DIRECTION ( 'NONE',  ( 0.000000000000000000, 1.000000000000000000, 0.000000000000000000 ) ) ;
#55932=EDGE_CURVE ( 'NONE', #101170, #8727, #48501, .T. ) ;
#55933=ORIENTED_EDGE ( 'NONE', *, *, #90615, .F. ) ;
#55934=LINE ( 'NONE', #127271, #126728 ) ;
#55935=PLANE ( 'NONE',  #15580 ) ;
#55936=VERTEX_POINT ( 'NONE', #89713 ) ;
#55937=CARTESIAN_POINT ( 'NONE',  ( 10.59999999999990905, 2.500000000000000000, 4.676537180435972552 ) ) ;
#55939=VERTEX_POINT ( 'NONE', #69416 ) ;
#55940=EDGE_CURVE ( 'NONE', #34057, #73263, #24101, .T. ) ;
#55941=DIRECTION ( 'NONE',  ( -0.000000000000000000, 1.000000000000000000, -0.000000000000000000 ) ) ;
#55942=AXIS2_PLACEMENT_3D ( 'NONE', #19189, #99072, #29681 ) ;
#55943=DIRECTION ( 'NONE',  ( -0.000000000000000000, 1.000000000000000000, -0.000000000000000000 ) ) ;
#55944=EDGE_LOOP ( 'NONE', ( #73735, #57890, #66484, #19142 ) ) ;
#55945=ORIENTED_EDGE ( 'NONE', *, *, #49431, .T. ) ;
#55946=CARTESIAN_POINT ( 'NONE',  ( 9.149999999999915090, 2.500000000000000000, -2.165063509461101710 ) ) ;
#55947=LINE ( 'NONE', #118089, #97357 ) ;
#55949=DIRECTION ( 'NONE',  ( 0.000000000000000000, 0.000000000000000000, 1.000000000000000000 ) ) ;
#55950=AXIS2_PLACEMENT_3D ( 'NONE', #107611, #125946, #56559 ) ;
#55952=DIRECTION ( 'NONE',  ( 0.000000000000000000, 1.000000000000000000, 0.000000000000000000 ) ) ;
#55953=CIRCLE ( 'NONE', #32990, 0.1000000000000002554 ) ;
#55955=ORIENTED_EDGE ( 'NONE', *, *, #46130, .T. ) ;
#55956=CARTESIAN_POINT ( 'NONE',  ( 4.149999999999941735, 2.500000000000000000, -7.288010851410854585 ) ) ;
#55957=ORIENTED_EDGE ( 'NONE', *, *, #6933, .F. ) ;
#55958=AXIS2_PLACEMENT_3D ( 'NONE', #74313, #84114, #124044 ) ;
#55959=DIRECTION ( 'NONE',  ( 0.000000000000000000, 0.000000000000000000, 1.000000000000000000 ) ) ;
#55960=CARTESIAN_POINT ( 'NONE',  ( 4.599999999999935696, 2.500000000000000000, 5.122947341949749323 ) ) ;
#55961=DIRECTION ( 'NONE',  ( 0.000000000000000000, 1.000000000000000000, 0.000000000000000000 ) ) ;
#55962=ORIENTED_EDGE ( 'NONE', *, *, #44811, .F. ) ;
#55963=AXIS2_PLACEMENT_3D ( 'NONE', #86255, #113313, #62925 ) ;
#55964=EDGE_CURVE ( 'NONE', #17990, #126026, #113980, .T. ) ;
#55965=DIRECTION ( 'NONE',  ( -4.274815082592931898E-19, -0.9999939076577903929, -0.003490651415223739937 ) ) ;
#55966=DIRECTION ( 'NONE',  ( -0.000000000000000000, 1.000000000000000000, -0.000000000000000000 ) ) ;
#55967=CONICAL_SURFACE ( 'NONE', #64292, 0.1000000000000002554, 0.003490658503988666988 ) ;
#55968=VERTEX_POINT ( 'NONE', #50431 ) ;
#55969=CONICAL_SURFACE ( 'NONE', #74862, 0.1000000000000002554, 0.003490658503988666988 ) ;
#55970=LINE ( 'NONE', #77543, #84423 ) ;
#55971=EDGE_CURVE ( 'NONE', #84309, #19348, #74280, .T. ) ;
#55972=VECTOR ( 'NONE', #76113, 1000.000000000000000 ) ;
#55973=VERTEX_POINT ( 'NONE', #118521 ) ;
#55974=ORIENTED_EDGE ( 'NONE', *, *, #104545, .T. ) ;
#55976=CONICAL_SURFACE ( 'NONE', #76919, 0.1000000000000002554, 0.003490658503988666988 ) ;
#55977=ORIENTED_EDGE ( 'NONE', *, *, #22308, .F. ) ;
#55978=CARTESIAN_POINT ( 'NONE',  ( 11.69999999999990870, 2.500000000000000000, -4.330127018922201643 ) ) ;
#55979=CARTESIAN_POINT ( 'NONE',  ( -14.79999999999998472, 2.500000000000000000, 0.2464101615137758439 ) ) ;
#55980=CIRCLE ( 'NONE', #10033, 0.1000000000000002554 ) ;
#55981=DIRECTION ( 'NONE',  ( 0.000000000000000000, 1.000000000000000000, 0.000000000000000000 ) ) ;
#55982=ORIENTED_EDGE ( 'NONE', *, *, #77544, .F. ) ;
#55983=CIRCLE ( 'NONE', #66452, 0.06509327318403745899 ) ;
#55984=FACE_BOUND ( 'NONE', #96430, .T. ) ;
#55985=DIRECTION ( 'NONE',  ( -4.274815082592931898E-19, -0.9999939076577903929, -0.003490651415223739937 ) ) ;
#55986=ORIENTED_EDGE ( 'NONE', *, *, #34968, .T. ) ;
#55987=FACE_OUTER_BOUND ( 'NONE', #21788, .T. ) ;
#55989=DIRECTION ( 'NONE',  ( -4.274815082592931898E-19, -0.9999939076577903929, -0.003490651415223739937 ) ) ;
#55990=ORIENTED_EDGE ( 'NONE', *, *, #102356, .T. ) ;
#55991=CIRCLE ( 'NONE', #72736, 0.06509327318403745899 ) ;
#55993=VERTEX_POINT ( 'NONE', #38036 ) ;
#55994=ORIENTED_EDGE ( 'NONE', *, *, #84735, .T. ) ;
#55995=CARTESIAN_POINT ( 'NONE',  ( -3.750000000000027534, 2.500000000000000000, -1.372243186433550033 ) ) ;
#55996=CARTESIAN_POINT ( 'NONE',  ( -8.550000000000011369, 2.500000000000000000, 1.818653347947321475 ) ) ;
#55997=CARTESIAN_POINT ( 'NONE',  ( 3.099999999999945022, 2.500000000000000000, -4.576537180435978236 ) ) ;
#55998=FACE_BOUND ( 'NONE', #44188, .T. ) ;
#55999=ORIENTED_EDGE ( 'NONE', *, *, #84164, .F. ) ;
#56001=LINE ( 'NONE', #105100, #44925 ) ;
#56002=DIRECTION ( 'NONE',  ( -0.000000000000000000, -1.000000000000000000, -0.000000000000000000 ) ) ;
#56003=ADVANCED_FACE ( 'NONE', ( #110007 ), #57892, .T. ) ;
#56005=CARTESIAN_POINT ( 'NONE',  ( -6.250000000000019540, 2.500000000000000000, -7.188010851410854052 ) ) ;
#56006=DIRECTION ( 'NONE',  ( 0.000000000000000000, 1.000000000000000000, 0.000000000000000000 ) ) ;
#56007=DIRECTION ( 'NONE',  ( 0.000000000000000000, 0.000000000000000000, 1.000000000000000000 ) ) ;
#56008=LINE ( 'NONE', #116861, #50267 ) ;
#56009=EDGE_CURVE ( 'NONE', #104853, #41663, #51311, .T. ) ;
#56010=CARTESIAN_POINT ( 'NONE',  ( -7.900000000000014566, 2.500000000000000000, -5.022947341949754119 ) ) ;
#56011=ORIENTED_EDGE ( 'NONE', *, *, #78930, .F. ) ;
#56012=EDGE_LOOP ( 'NONE', ( #78378, #49325 ) ) ;
#56013=ORIENTED_EDGE ( 'NONE', *, *, #50466, .T. ) ;
#56014=VERTEX_POINT ( 'NONE', #58971 ) ;
#56015=ORIENTED_EDGE ( 'NONE', *, *, #34862, .F. ) ;
#56017=AXIS2_PLACEMENT_3D ( 'NONE', #50262, #129489, #118991 ) ;
#56018=ADVANCED_FACE ( 'NONE', ( #681 ), #68128, .T. ) ;
#56019=CARTESIAN_POINT ( 'NONE',  ( -15.39999999999998082, 2.500000000000000000, 0.7928203230275517877 ) ) ;
#56020=ORIENTED_EDGE ( 'NONE', *, *, #81163, .T. ) ;
#56021=FACE_BOUND ( 'NONE', #53370, .T. ) ;
#56022=EDGE_CURVE ( 'NONE', #118638, #26544, #30710, .T. ) ;
#56023=LINE ( 'NONE', #126056, #83486 ) ;
#56024=CONICAL_SURFACE ( 'NONE', #45583, 0.09999999999999999167, 0.003490658503988666988 ) ;
#56025=VECTOR ( 'NONE', #70161, 1000.000000000000000 ) ;
#56026=EDGE_CURVE ( 'NONE', #94402, #96192, #9846, .T. ) ;
#56027=LINE ( 'NONE', #54733, #5092 ) ;
#56028=DIRECTION ( 'NONE',  ( 0.000000000000000000, 0.000000000000000000, 1.000000000000000000 ) ) ;
#56030=ADVANCED_FACE ( 'NONE', ( #88408 ), #49574, .T. ) ;
#56031=DIRECTION ( 'NONE',  ( 0.000000000000000000, 1.000000000000000000, 0.000000000000000000 ) ) ;
#56033=CONICAL_SURFACE ( 'NONE', #70714, 0.1000000000000002554, 0.003490658503988666988 ) ;
#56034=ORIENTED_EDGE ( 'NONE', *, *, #125476, .T. ) ;
#56035=CIRCLE ( 'NONE', #102025, 0.06509327318403745899 ) ;
#56036=EDGE_LOOP ( 'NONE', ( #121779, #14802 ) ) ;
#56037=EDGE_LOOP ( 'NONE', ( #9512, #81616 ) ) ;
#56038=CARTESIAN_POINT ( 'NONE',  ( -9.800000000000006040, 12.50000000000000000, -4.676537180435974328 ) ) ;
#56040=DIRECTION ( 'NONE',  ( 0.000000000000000000, 0.000000000000000000, 1.000000000000000000 ) ) ;
#56041=ORIENTED_EDGE ( 'NONE', *, *, #16988, .T. ) ;
#56042=DIRECTION ( 'NONE',  ( -0.000000000000000000, 1.000000000000000000, -0.000000000000000000 ) ) ;
#56043=CONICAL_SURFACE ( 'NONE', #129251, 0.1000000000000002554, 0.003490658503988666988 ) ;
#56044=DIRECTION ( 'NONE',  ( 0.000000000000000000, 1.000000000000000000, 0.000000000000000000 ) ) ;
#56045=LINE ( 'NONE', #124807, #30690 ) ;
#56047=FACE_OUTER_BOUND ( 'NONE', #84836, .T. ) ;
#56048=AXIS2_PLACEMENT_3D ( 'NONE', #58395, #47280, #47926 ) ;
#56049=CARTESIAN_POINT ( 'NONE',  ( -11.05000000000000071, 12.50000000000000000, 6.906693963081109722 ) ) ;
#56051=FACE_OUTER_BOUND ( 'NONE', #38295, .T. ) ;
#56052=CIRCLE ( 'NONE', #60302, 0.06509327318403745899 ) ;
#56053=EDGE_LOOP ( 'NONE', ( #110746, #67034 ) ) ;
#56054=EDGE_LOOP ( 'NONE', ( #4205, #31380 ) ) ;
#56055=AXIS2_PLACEMENT_3D ( 'NONE', #10036, #29044, #37571 ) ;
#56056=CARTESIAN_POINT ( 'NONE',  ( -11.44999999999999929, 12.50000000000000000, -1.818653347947322141 ) ) ;
#56057=DIRECTION ( 'NONE',  ( 0.000000000000000000, 1.000000000000000000, 0.000000000000000000 ) ) ;
#56058=CARTESIAN_POINT ( 'NONE',  ( 2.899999999999946620, 2.500000000000000000, -0.6928203230275542523 ) ) ;
#56059=CIRCLE ( 'NONE', #64383, 0.06509327318403741736 ) ;
#56060=ORIENTED_EDGE ( 'NONE', *, *, #45605, .F. ) ;
#56061=CIRCLE ( 'NONE', #62444, 0.06509327318403745899 ) ;
#56062=EDGE_LOOP ( 'NONE', ( #67850, #53791 ) ) ;
#56063=ADVANCED_FACE ( 'NONE', ( #79267 ), #28876, .T. ) ;
#56064=CARTESIAN_POINT ( 'NONE',  ( 3.149999999999946176, 2.500000000000000000, -1.718653347947325827 ) ) ;
#56065=AXIS2_PLACEMENT_3D ( 'NONE', #117954, #126504, #37492 ) ;
#56066=DIRECTION ( 'NONE',  ( 0.000000000000000000, -0.9999939076577903929, 0.003490651415223739937 ) ) ;
#56067=DIRECTION ( 'NONE',  ( -4.274815082592931898E-19, -0.9999939076577903929, -0.003490651415223739937 ) ) ;
#56068=EDGE_CURVE ( 'NONE', #125967, #72978, #101800, .T. ) ;
#56069=EDGE_LOOP ( 'NONE', ( #15416, #19382, #16716, #68072 ) ) ;
#56070=VERTEX_POINT ( 'NONE', #113207 ) ;
#56071=EDGE_CURVE ( 'NONE', #92620, #66161, #72559, .T. ) ;
#56072=DIRECTION ( 'NONE',  ( 0.000000000000000000, -0.9999939076577903929, 0.003490651415223739937 ) ) ;
#56073=CIRCLE ( 'NONE', #68596, 0.1000000000000002554 ) ;
#56074=EDGE_CURVE ( 'NONE', #58451, #73869, #70399, .T. ) ;
#56075=EDGE_CURVE ( 'NONE', #27855, #64286, #99749, .T. ) ;
#56076=VERTEX_POINT ( 'NONE', #31450 ) ;
#56077=DIRECTION ( 'NONE',  ( -0.000000000000000000, 1.000000000000000000, -0.000000000000000000 ) ) ;
#56078=CARTESIAN_POINT ( 'NONE',  ( -8.950000000000011724, 2.500000000000000000, -6.148780366869520897 ) ) ;
#56079=EDGE_LOOP ( 'NONE', ( #27913, #87203, #121550, #119355 ) ) ;
#56080=DIRECTION ( 'NONE',  ( 0.000000000000000000, 1.000000000000000000, 0.000000000000000000 ) ) ;
#56081=EDGE_CURVE ( 'NONE', #128794, #105778, #97576, .T. ) ;
#56082=DIRECTION ( 'NONE',  ( 0.000000000000000000, -0.9999939076577903929, 0.003490651415223739937 ) ) ;
#56083=DIRECTION ( 'NONE',  ( 0.000000000000000000, 0.000000000000000000, 1.000000000000000000 ) ) ;
#56084=AXIS2_PLACEMENT_3D ( 'NONE', #26732, #106570, #117657 ) ;
#56085=CARTESIAN_POINT ( 'NONE',  ( 10.64999999999990976, 12.50000000000000000, 1.883746621131358934 ) ) ;
#56086=ORIENTED_EDGE ( 'NONE', *, *, #67123, .T. ) ;
#56087=EDGE_CURVE ( 'NONE', #111256, #19044, #11895, .T. ) ;
#56088=CARTESIAN_POINT ( 'NONE',  ( -0.8500000000000390576, 2.500000000000000000, -6.495190528383302464 ) ) ;
#56089=CIRCLE ( 'NONE', #53957, 0.06509327318403745899 ) ;
#56090=EDGE_CURVE ( 'NONE', #59007, #16781, #123048, .T. ) ;
#56091=LINE ( 'NONE', #32405, #45736 ) ;
#56092=EDGE_LOOP ( 'NONE', ( #128608, #31077, #108898, #114075 ) ) ;
#56093=VERTEX_POINT ( 'NONE', #110639 ) ;
#56095=DIRECTION ( 'NONE',  ( -0.000000000000000000, -1.000000000000000000, -0.000000000000000000 ) ) ;
#56096=PLANE ( 'NONE',  #84497 ) ;
#56097=FACE_OUTER_BOUND ( 'NONE', #115776, .T. ) ;
#56098=CARTESIAN_POINT ( 'NONE',  ( -12.49999999999999467, 2.500000000000000000, -3.537306695894647302 ) ) ;
#56099=CARTESIAN_POINT ( 'NONE',  ( 8.549999999999918998, 12.50000000000000000, -1.818653347947326138 ) ) ;
#56100=CARTESIAN_POINT ( 'NONE',  ( 5.449999999999937117, 12.50000000000000000, -6.430097255199264339 ) ) ;
#56101=CARTESIAN_POINT ( 'NONE',  ( -6.050000000000022027, 2.500000000000000000, -6.248780366869526759 ) ) ;
#56102=CARTESIAN_POINT ( 'NONE',  ( -3.350000000000028955, 12.50000000000000000, 7.188010851410848723 ) ) ;
#56103=AXIS2_PLACEMENT_3D ( 'NONE', #121705, #71313, #71983 ) ;
#56104=CARTESIAN_POINT ( 'NONE',  ( 10.64999999999991331, 2.500000000000000000, -2.511473670974877948 ) ) ;
#56105=VERTEX_POINT ( 'NONE', #111257 ) ;
#56106=CIRCLE ( 'NONE', #119100, 7.500000000000000000 ) ;
#56107=CONICAL_SURFACE ( 'NONE', #72852, 0.1000000000000002554, 0.003490658503988666988 ) ;
#56108=ORIENTED_EDGE ( 'NONE', *, *, #127435, .T. ) ;
#56109=AXIS2_PLACEMENT_3D ( 'NONE', #4376, #44990, #66539 ) ;
#56110=DIRECTION ( 'NONE',  ( 0.000000000000000000, 1.000000000000000000, 0.000000000000000000 ) ) ;
#56111=VERTEX_POINT ( 'NONE', #102117 ) ;
#56112=DIRECTION ( 'NONE',  ( 0.000000000000000000, -0.000000000000000000, 1.000000000000000000 ) ) ;
#56113=DIRECTION ( 'NONE',  ( -0.000000000000000000, -1.000000000000000000, -0.000000000000000000 ) ) ;
#56114=CARTESIAN_POINT ( 'NONE',  ( 11.24999999999991118, 2.500000000000000000, 5.802370205355744659 ) ) ;
#56115=AXIS2_PLACEMENT_3D ( 'NONE', #22605, #90673, #111606 ) ;
#56116=EDGE_LOOP ( 'NONE', ( #53926, #51583 ) ) ;
#56117=AXIS2_PLACEMENT_3D ( 'NONE', #53675, #15006, #43875 ) ;
#56118=CARTESIAN_POINT ( 'NONE',  ( -14.14999999999998614, 12.50000000000000000, -2.165063509461099489 ) ) ;
#56119=VECTOR ( 'NONE', #82989, 1000.000000000000000 ) ;
#56120=CARTESIAN_POINT ( 'NONE',  ( 7.499999999999960032, 2.500000000000000000, 0.09999999999999772959 ) ) ;
#56121=CARTESIAN_POINT ( 'NONE',  ( 13.29999999999990301, 12.50000000000000000, 4.330127018922196314 ) ) ;
#56122=ORIENTED_EDGE ( 'NONE', *, *, #8470, .F. ) ;
#56123=AXIS2_PLACEMENT_3D ( 'NONE', #87547, #38484, #109780 ) ;
#56124=CARTESIAN_POINT ( 'NONE',  ( 4.799999999999937650, 2.500000000000000000, -4.083716857408426826 ) ) ;
#56125=ORIENTED_EDGE ( 'NONE', *, *, #23212, .F. ) ;
#56126=EDGE_CURVE ( 'NONE', #120581, #63587, #47424, .T. ) ;
#56127=AXIS2_PLACEMENT_3D ( 'NONE', #100854, #11188, #71391 ) ;
#56128=VERTEX_POINT ( 'NONE', #12429 ) ;
#56129=EDGE_LOOP ( 'NONE', ( #51192, #119662 ) ) ;
#56130=VERTEX_POINT ( 'NONE', #33392 ) ;
#56131=LINE ( 'NONE', #113785, #119988 ) ;
#56132=DIRECTION ( 'NONE',  ( 0.000000000000000000, 0.000000000000000000, 1.000000000000000000 ) ) ;
#56133=CARTESIAN_POINT ( 'NONE',  ( 3.299999999999942979, 12.50000000000000000, 4.330127018922196314 ) ) ;
#56134=CARTESIAN_POINT ( 'NONE',  ( -8.350000000000012079, 2.500000000000000000, 1.472243186433545459 ) ) ;
#56135=CIRCLE ( 'NONE', #47652, 0.06509327318403745899 ) ;
#56136=VERTEX_POINT ( 'NONE', #41916 ) ;
#56138=DIRECTION ( 'NONE',  ( 0.000000000000000000, 0.000000000000000000, 1.000000000000000000 ) ) ;
#56139=VERTEX_POINT ( 'NONE', #22916 ) ;
#56140=AXIS2_PLACEMENT_3D ( 'NONE', #126155, #75122, #5080 ) ;
#56141=DIRECTION ( 'NONE',  ( 0.000000000000000000, -0.000000000000000000, -1.000000000000000000 ) ) ;
#56142=DIRECTION ( 'NONE',  ( 0.000000000000000000, 0.000000000000000000, 1.000000000000000000 ) ) ;
#56143=FACE_OUTER_BOUND ( 'NONE', #14911, .T. ) ;
#56144=CARTESIAN_POINT ( 'NONE',  ( 20.69433222467931444, -2.585316282066745242, 4.139109617385087425 ) ) ;
#56145=VERTEX_POINT ( 'NONE', #83130 ) ;
#56146=AXIS2_PLACEMENT_3D ( 'NONE', #83652, #63362, #103293 ) ;
#56148=ORIENTED_EDGE ( 'NONE', *, *, #52542, .F. ) ;
#56149=EDGE_LOOP ( 'NONE', ( #13805, #19063, #109917, #40795 ) ) ;
#56150=CARTESIAN_POINT ( 'NONE',  ( 1.049999999999954525, 12.50000000000000000, -2.511473670974877948 ) ) ;
#56151=LINE ( 'NONE', #96087, #14266 ) ;
#56152=DIRECTION ( 'NONE',  ( -0.000000000000000000, -1.000000000000000000, -0.000000000000000000 ) ) ;
#56153=FACE_BOUND ( 'NONE', #97108, .T. ) ;
#56154=FACE_OUTER_BOUND ( 'NONE', #80344, .T. ) ;
#56155=DIRECTION ( 'NONE',  ( 0.000000000000000000, 1.000000000000000000, 0.000000000000000000 ) ) ;
#56156=AXIS2_PLACEMENT_3D ( 'NONE', #97143, #68319, #7458 ) ;
#56157=DIRECTION ( 'NONE',  ( 0.000000000000000000, -0.000000000000000000, 1.000000000000000000 ) ) ;
#56158=FACE_OUTER_BOUND ( 'NONE', #12225, .T. ) ;
#56159=CIRCLE ( 'NONE', #110546, 0.1000000000000002554 ) ;
#56161=DIRECTION ( 'NONE',  ( -4.274815082592931898E-19, -0.9999939076577903929, -0.003490651415223739937 ) ) ;
#56162=CIRCLE ( 'NONE', #35264, 0.1000000000000000472 ) ;
#56163=DIRECTION ( 'NONE',  ( -0.000000000000000000, 1.000000000000000000, -0.000000000000000000 ) ) ;
#56164=EDGE_CURVE ( 'NONE', #50689, #18883, #60894, .T. ) ;
#56165=DIRECTION ( 'NONE',  ( 0.000000000000000000, 0.000000000000000000, -1.000000000000000000 ) ) ;
#56166=AXIS2_PLACEMENT_3D ( 'NONE', #75311, #97528, #56941 ) ;
#56167=VERTEX_POINT ( 'NONE', #93584 ) ;
#56168=EDGE_LOOP ( 'NONE', ( #113014, #79162, #41762, #123618 ) ) ;
#56169=VERTEX_POINT ( 'NONE', #32750 ) ;
#56170=ORIENTED_EDGE ( 'NONE', *, *, #71914, .F. ) ;
#56172=CARTESIAN_POINT ( 'NONE',  ( 9.349999999999916156, 2.500000000000000000, 6.248780366869520542 ) ) ;
#56173=FACE_BOUND ( 'NONE', #60042, .T. ) ;
#56174=EDGE_CURVE ( 'NONE', #12327, #30034, #112265, .T. ) ;
#56175=DIRECTION ( 'NONE',  ( -0.000000000000000000, -1.000000000000000000, -0.000000000000000000 ) ) ;
#56176=DIRECTION ( 'NONE',  ( -0.000000000000000000, -1.000000000000000000, -0.000000000000000000 ) ) ;
#56177=VECTOR ( 'NONE', #11010, 1000.000000000000000 ) ;
#56178=AXIS2_PLACEMENT_3D ( 'NONE', #67215, #16828, #26690 ) ;
#56179=ADVANCED_FACE ( 'NONE', ( #102741 ), #68338, .T. ) ;
#56180=ADVANCED_FACE ( 'NONE', ( #91006 ), #55817, .T. ) ;
#56181=ORIENTED_EDGE ( 'NONE', *, *, #72468, .T. ) ;
#56182=DIRECTION ( 'NONE',  ( 0.000000000000000000, -0.000000000000000000, 1.000000000000000000 ) ) ;
#56183=ADVANCED_FACE ( 'NONE', ( #3270 ), #111940, .T. ) ;
#56184=DIRECTION ( 'NONE',  ( 0.000000000000000000, 1.000000000000000000, 0.000000000000000000 ) ) ;
#56185=ADVANCED_FACE ( 'NONE', ( #91646 ), #1965, .T. ) ;
#56186=EDGE_LOOP ( 'NONE', ( #107460, #91354, #35188, #68340 ) ) ;
#56187=CARTESIAN_POINT ( 'NONE',  ( -6.505213034913026604E-15, 2.500000000000000000, 4.430127018922196847 ) ) ;
#56188=DIRECTION ( 'NONE',  ( -0.000000000000000000, 1.000000000000000000, -0.000000000000000000 ) ) ;
#56189=ORIENTED_EDGE ( 'NONE', *, *, #55152, .F. ) ;
#56190=AXIS2_PLACEMENT_3D ( 'NONE', #45740, #36578, #47035 ) ;
#56191=CARTESIAN_POINT ( 'NONE',  ( -12.94999999999999218, 12.50000000000000000, 2.165063509461101265 ) ) ;
#56192=DIRECTION ( 'NONE',  ( 0.000000000000000000, 0.000000000000000000, -1.000000000000000000 ) ) ;
#56193=ADVANCED_FACE ( 'NONE', ( #7116 ), #59966, .T. ) ;
#56194=ORIENTED_EDGE ( 'NONE', *, *, #29482, .T. ) ;
#56195=VECTOR ( 'NONE', #117122, 1000.000000000000000 ) ;
#56196=DIRECTION ( 'NONE',  ( 0.000000000000000000, 0.000000000000000000, 1.000000000000000000 ) ) ;
#56197=CIRCLE ( 'NONE', #12286, 0.06509327318403741736 ) ;
#56198=CARTESIAN_POINT ( 'NONE',  ( 7.099999999999926814, 12.50000000000000000, -0.6928203230275541413 ) ) ;
#56199=ORIENTED_EDGE ( 'NONE', *, *, #43095, .T. ) ;
#56200=DIRECTION ( 'NONE',  ( 0.000000000000000000, 0.000000000000000000, 1.000000000000000000 ) ) ;
#56201=EDGE_LOOP ( 'NONE', ( #14776, #103589 ) ) ;
#56202=EDGE_LOOP ( 'NONE', ( #85358, #80108 ) ) ;
#56203=DIRECTION ( 'NONE',  ( 0.000000000000000000, 0.000000000000000000, 1.000000000000000000 ) ) ;
#56204=VECTOR ( 'NONE', #110845, 1000.000000000000000 ) ;
#56205=VERTEX_POINT ( 'NONE', #4521 ) ;
#56206=CARTESIAN_POINT ( 'NONE',  ( -0.2000000000000404232, 12.50000000000000000, 3.983716857408420964 ) ) ;
#56207=CARTESIAN_POINT ( 'NONE',  ( 6.449999999999933564, 2.500000000000000000, -6.841600689897078702 ) ) ;
#56208=AXIS2_PLACEMENT_3D ( 'NONE', #101985, #79756, #12294 ) ;
#56209=ORIENTED_EDGE ( 'NONE', *, *, #83826, .T. ) ;
#56210=CARTESIAN_POINT ( 'NONE',  ( 0.8499999999999550138, 12.50000000000000000, -5.802370205355749988 ) ) ;
#56211=FACE_OUTER_BOUND ( 'NONE', #30632, .T. ) ;
#56212=CARTESIAN_POINT ( 'NONE',  ( 10.59999999999990905, 2.500000000000000000, 4.083716857408420609 ) ) ;
#56214=EDGE_CURVE ( 'NONE', #94677, #8342, #41179, .T. ) ;
#56215=CARTESIAN_POINT ( 'NONE',  ( -8.750000000000008882, 2.500000000000000000, -2.857883832488653741 ) ) ;
#56216=DIRECTION ( 'NONE',  ( -0.000000000000000000, -1.000000000000000000, -0.000000000000000000 ) ) ;
#56217=AXIS2_PLACEMENT_3D ( 'NONE', #13491, #124749, #14137 ) ;
#56218=VERTEX_POINT ( 'NONE', #54933 ) ;
#56219=AXIS2_PLACEMENT_3D ( 'NONE', #94760, #43755, #3804 ) ;
#56220=ORIENTED_EDGE ( 'NONE', *, *, #46316, .F. ) ;
#56221=DIRECTION ( 'NONE',  ( -0.000000000000000000, -1.000000000000000000, -0.000000000000000000 ) ) ;
#56222=DIRECTION ( 'NONE',  ( 0.000000000000000000, 0.000000000000000000, 1.000000000000000000 ) ) ;
#56223=FACE_OUTER_BOUND ( 'NONE', #95994, .T. ) ;
#56224=EDGE_CURVE ( 'NONE', #81996, #20105, #78829, .T. ) ;
#56225=EDGE_LOOP ( 'NONE', ( #106936, #45975, #4885, #47615 ) ) ;
#56226=ORIENTED_EDGE ( 'NONE', *, *, #97191, .F. ) ;
#56227=ORIENTED_EDGE ( 'NONE', *, *, #54546, .T. ) ;
#56228=ADVANCED_FACE ( 'NONE', ( #64755 ), #93385, .T. ) ;
#56229=DIRECTION ( 'NONE',  ( -0.000000000000000000, 1.000000000000000000, -0.000000000000000000 ) ) ;
#56231=CIRCLE ( 'NONE', #89410, 0.06509327318403745899 ) ;
#56232=DIRECTION ( 'NONE',  ( -0.000000000000000000, -1.000000000000000000, -0.000000000000000000 ) ) ;
#56233=DIRECTION ( 'NONE',  ( 0.000000000000000000, 1.000000000000000000, 0.000000000000000000 ) ) ;
#56234=EDGE_CURVE ( 'NONE', #1556, #125732, #115121, .T. ) ;
#56236=CARTESIAN_POINT ( 'NONE',  ( -12.89999999999999325, 2.500000000000000000, -3.537306695894647302 ) ) ;
#56237=DIRECTION ( 'NONE',  ( -0.000000000000000000, -1.000000000000000000, -0.000000000000000000 ) ) ;
#56239=FACE_OUTER_BOUND ( 'NONE', #100566, .T. ) ;
#56240=AXIS2_PLACEMENT_3D ( 'NONE', #27725, #27097, #36287 ) ;
#56241=FACE_OUTER_BOUND ( 'NONE', #57042, .T. ) ;
#56242=ADVANCED_FACE ( 'NONE', ( #95518 ), #104670, .T. ) ;
#56243=CARTESIAN_POINT ( 'NONE',  ( -9.350000000000006750, 2.500000000000000000, 2.611473670974873151 ) ) ;
#56244=ADVANCED_FACE ( 'NONE', ( #47070 ), #74603, .T. ) ;
#56245=ADVANCED_FACE ( 'NONE', ( #14986 ), #122722, .T. ) ;
#56246=EDGE_LOOP ( 'NONE', ( #25767, #101916 ) ) ;
#56247=ADVANCED_FACE ( 'NONE', ( #125600 ), #75224, .T. ) ;
#56248=AXIS2_PLACEMENT_3D ( 'NONE', #89432, #99905, #128743 ) ;
#56249=CARTESIAN_POINT ( 'NONE',  ( 10.44999999999991402, 12.50000000000000000, -2.230156782645139391 ) ) ;
#56250=VERTEX_POINT ( 'NONE', #96783 ) ;
#56251=EDGE_LOOP ( 'NONE', ( #61672, #31455, #95750, #10937 ) ) ;
#56252=DIRECTION ( 'NONE',  ( 0.000000000000000000, 1.000000000000000000, 0.000000000000000000 ) ) ;
#56253=DIRECTION ( 'NONE',  ( -0.000000000000000000, -1.000000000000000000, -0.000000000000000000 ) ) ;
#56254=AXIS2_PLACEMENT_3D ( 'NONE', #114684, #64933, #85234 ) ;
#56255=DIRECTION ( 'NONE',  ( 0.000000000000000000, 0.000000000000000000, 1.000000000000000000 ) ) ;
#56256=ADVANCED_FACE ( 'NONE', ( #5180 ), #36958, .T. ) ;
#56257=FACE_OUTER_BOUND ( 'NONE', #50579, .T. ) ;
#56258=VECTOR ( 'NONE', #126013, 1000.000000000000000 ) ;
#56260=DIRECTION ( 'NONE',  ( -0.000000000000000000, -1.000000000000000000, -0.000000000000000000 ) ) ;
#56261=LINE ( 'NONE', #96179, #57294 ) ;
#56262=VERTEX_POINT ( 'NONE', #94868 ) ;
#56263=CARTESIAN_POINT ( 'NONE',  ( 10.39999999999990976, 12.50000000000000000, -4.395220292106239768 ) ) ;
#56264=AXIS2_PLACEMENT_3D ( 'NONE', #125115, #15791, #36095 ) ;
#56265=DIRECTION ( 'NONE',  ( 0.000000000000000000, -0.000000000000000000, 1.000000000000000000 ) ) ;
#56266=ORIENTED_EDGE ( 'NONE', *, *, #74731, .F. ) ;
#56267=VERTEX_POINT ( 'NONE', #14357 ) ;
#56268=CIRCLE ( 'NONE', #127297, 0.06509327318403745899 ) ;
#56269=CONICAL_SURFACE ( 'NONE', #121025, 0.1000000000000000472, 0.003490658503988666988 ) ;
#56270=ORIENTED_EDGE ( 'NONE', *, *, #30073, .T. ) ;
#56271=CONICAL_SURFACE ( 'NONE', #66730, 0.1000000000000000472, 0.003490658503988666988 ) ;
#56272=ORIENTED_EDGE ( 'NONE', *, *, #33484, .F. ) ;
#56273=CARTESIAN_POINT ( 'NONE',  ( 9.149999999999916866, 12.50000000000000000, -2.922977105672691422 ) ) ;
#56274=CARTESIAN_POINT ( 'NONE',  ( 1.049999999999952083, 2.500000000000000000, 6.841600689897072485 ) ) ;
#56275=AXIS2_PLACEMENT_3D ( 'NONE', #72423, #101877, #103158 ) ;
#56276=DIRECTION ( 'NONE',  ( 0.000000000000000000, 0.000000000000000000, -1.000000000000000000 ) ) ;
#56277=CARTESIAN_POINT ( 'NONE',  ( 17.50000000000000000, 0.9166666666666682950, -3.999999999999998224 ) ) ;
#56278=DIRECTION ( 'NONE',  ( -0.000000000000000000, -1.000000000000000000, -0.000000000000000000 ) ) ;
#56279=ORIENTED_EDGE ( 'NONE', *, *, #93295, .T. ) ;
#56280=CARTESIAN_POINT ( 'NONE',  ( -1.250000000000037526, 2.500000000000000000, -1.472243186433550122 ) ) ;
#56281=CARTESIAN_POINT ( 'NONE',  ( -8.550000000000013145, 2.500000000000000000, -1.718653347947326049 ) ) ;
#56282=ORIENTED_EDGE ( 'NONE', *, *, #80124, .T. ) ;
#56283=EDGE_CURVE ( 'NONE', #28419, #122300, #91324, .T. ) ;
#56284=ORIENTED_EDGE ( 'NONE', *, *, #115591, .F. ) ;
#56285=VERTEX_POINT ( 'NONE', #34682 ) ;
#56286=VECTOR ( 'NONE', #97097, 1000.000000000000000 ) ;
#56287=DIRECTION ( 'NONE',  ( 0.000000000000000000, 0.000000000000000000, 1.000000000000000000 ) ) ;
#56288=DIRECTION ( 'NONE',  ( -0.000000000000000000, 1.000000000000000000, -0.000000000000000000 ) ) ;
#56289=VECTOR ( 'NONE', #33919, 1000.000000000000000 ) ;
#56291=ORIENTED_EDGE ( 'NONE', *, *, #13608, .F. ) ;
#56292=DIRECTION ( 'NONE',  ( 0.000000000000000000, 1.000000000000000000, 0.000000000000000000 ) ) ;
#56293=CARTESIAN_POINT ( 'NONE',  ( -4.077824815344644402E-14, 2.500000000000000000, -5.122947341949753763 ) ) ;
#56294=ADVANCED_FACE ( 'NONE', ( #44473 ), #66373, .T. ) ;
#56295=CARTESIAN_POINT ( 'NONE',  ( 8.549999999999924327, 2.500000000000000000, 1.818653347947321475 ) ) ;
#56296=DIRECTION ( 'NONE',  ( -0.000000000000000000, -1.000000000000000000, -0.000000000000000000 ) ) ;
#56297=AXIS2_PLACEMENT_3D ( 'NONE', #26357, #64966, #37470 ) ;
#56298=CONICAL_SURFACE ( 'NONE', #24920, 0.1000000000000002554, 0.003490658503988666988 ) ;
#56299=VERTEX_POINT ( 'NONE', #126266 ) ;
#56300=AXIS2_PLACEMENT_3D ( 'NONE', #85841, #76039, #116593 ) ;
#56301=CARTESIAN_POINT ( 'NONE',  ( 7.099999999999928590, 12.50000000000000000, 3.637306695894644726 ) ) ;
#56302=EDGE_LOOP ( 'NONE', ( #37693, #43897 ) ) ;
#56303=EDGE_LOOP ( 'NONE', ( #43855, #85500, #52463, #36844 ) ) ;
#56304=ORIENTED_EDGE ( 'NONE', *, *, #53272, .F. ) ;
#56305=DIRECTION ( 'NONE',  ( -0.000000000000000000, 1.000000000000000000, -0.000000000000000000 ) ) ;
#56306=FACE_BOUND ( 'NONE', #12812, .T. ) ;
#56307=AXIS2_PLACEMENT_3D ( 'NONE', #90613, #111549, #62473 ) ;
#56308=CARTESIAN_POINT ( 'NONE',  ( -13.34999999999999076, 12.50000000000000000, 1.472243186433549456 ) ) ;
#56310=DIRECTION ( 'NONE',  ( 0.000000000000000000, 0.000000000000000000, -1.000000000000000000 ) ) ;
#56311=AXIS2_PLACEMENT_3D ( 'NONE', #114091, #94435, #83969 ) ;
#56312=AXIS2_PLACEMENT_3D ( 'NONE', #48601, #46665, #40069 ) ;
#56313=ORIENTED_EDGE ( 'NONE', *, *, #19435, .T. ) ;
#56314=PLANE ( 'NONE',  #79800 ) ;
#56315=CARTESIAN_POINT ( 'NONE',  ( 1.649999999999951061, 12.50000000000000000, -6.495190528383302464 ) ) ;
#56316=DIRECTION ( 'NONE',  ( -0.000000000000000000, 1.000000000000000000, -0.000000000000000000 ) ) ;
#56317=CARTESIAN_POINT ( 'NONE',  ( -1.650000000000034328, 2.500000000000000000, -2.857883832488653741 ) ) ;
#56318=ORIENTED_EDGE ( 'NONE', *, *, #24924, .F. ) ;
#56319=CARTESIAN_POINT ( 'NONE',  ( -1.900000000000034994, 2.500000000000000000, -4.676537180435978769 ) ) ;
#56320=ADVANCED_FACE ( 'NONE', ( #36616 ), #51715, .T. ) ;
#56321=DIRECTION ( 'NONE',  ( 0.000000000000000000, 1.000000000000000000, 0.000000000000000000 ) ) ;
#56322=CIRCLE ( 'NONE', #73246, 0.06509327318403745899 ) ;
#56323=ORIENTED_EDGE ( 'NONE', *, *, #5112, .T. ) ;
#56324=FACE_OUTER_BOUND ( 'NONE', #57555, .T. ) ;
#56325=FACE_BOUND ( 'NONE', #59472, .T. ) ;
#56326=EDGE_CURVE ( 'NONE', #32792, #51798, #74585, .T. ) ;
#56327=FACE_OUTER_BOUND ( 'NONE', #127407, .T. ) ;
#56328=EDGE_LOOP ( 'NONE', ( #99953, #102247, #102392, #66458 ) ) ;
#56329=CARTESIAN_POINT ( 'NONE',  ( -3.150000000000029665, 2.500000000000000000, 6.841600689897072485 ) ) ;
#56330=DIRECTION ( 'NONE',  ( -0.000000000000000000, 1.000000000000000000, -0.000000000000000000 ) ) ;
#56331=EDGE_CURVE ( 'NONE', #28423, #2568, #3676, .T. ) ;
#56332=ORIENTED_EDGE ( 'NONE', *, *, #55767, .F. ) ;
#56333=EDGE_CURVE ( 'NONE', #104821, #127509, #83111, .T. ) ;
#56334=ORIENTED_EDGE ( 'NONE', *, *, #54461, .F. ) ;
#56336=EDGE_CURVE ( 'NONE', #10701, #109829, #118598, .T. ) ;
#56337=ADVANCED_FACE ( 'NONE', ( #119655 ), #11995, .T. ) ;
#56339=ADVANCED_FACE ( 'NONE', ( #27394 ), #67304, .T. ) ;
#56340=VERTEX_POINT ( 'NONE', #60125 ) ;
#56342=CARTESIAN_POINT ( 'NONE',  ( -7.100000000000018296, 12.50000000000000000, -4.265033745738164406 ) ) ;
#56343=CARTESIAN_POINT ( 'NONE',  ( 1.249999999999988454, 2.500000000000000000, 2.065063509461097624 ) ) ;
#56344=LINE ( 'NONE', #60083, #25926 ) ;
#56345=CARTESIAN_POINT ( 'NONE',  ( 8.099999999999921485, 2.500000000000000000, 0.4464101615137735513 ) ) ;
#56346=AXIS2_PLACEMENT_3D ( 'NONE', #30340, #39524, #121276 ) ;
#56347=ADVANCED_FACE ( 'NONE', ( #47714 ), #91411, .T. ) ;
#56348=ADVANCED_FACE ( 'NONE', ( #87615 ), #30009, .T. ) ;
#56349=ADVANCED_FACE ( 'NONE', ( #37253 ), #76750, .T. ) ;
#56350=VERTEX_POINT ( 'NONE', #126916 ) ;
#56351=DIRECTION ( 'NONE',  ( 0.000000000000000000, 0.000000000000000000, -1.000000000000000000 ) ) ;
#56352=AXIS2_PLACEMENT_3D ( 'NONE', #107147, #28611, #17471 ) ;
#56353=DIRECTION ( 'NONE',  ( 0.000000000000000000, -0.9999939076577903929, 0.003490651415223739937 ) ) ;
#56354=DIRECTION ( 'NONE',  ( 0.000000000000000000, -0.9999939076577903929, 0.003490651415223739937 ) ) ;
#56355=DIRECTION ( 'NONE',  ( -4.274815082592931898E-19, -0.9999939076577903929, -0.003490651415223739937 ) ) ;
#56356=AXIS2_PLACEMENT_3D ( 'NONE', #87898, #68269, #57824 ) ;
#56357=ORIENTED_EDGE ( 'NONE', *, *, #9231, .T. ) ;
#56358=ORIENTED_EDGE ( 'NONE', *, *, #26004, .T. ) ;
#56359=FACE_BOUND ( 'NONE', #43598, .T. ) ;
#56360=ORIENTED_EDGE ( 'NONE', *, *, #123838, .F. ) ;
#56361=FACE_OUTER_BOUND ( 'NONE', #5827, .T. ) ;
#56362=DIRECTION ( 'NONE',  ( -0.000000000000000000, 1.000000000000000000, -0.000000000000000000 ) ) ;
#56363=ORIENTED_EDGE ( 'NONE', *, *, #52533, .F. ) ;
#56364=DIRECTION ( 'NONE',  ( 0.000000000000000000, 0.000000000000000000, 1.000000000000000000 ) ) ;
#56366=AXIS2_PLACEMENT_3D ( 'NONE', #81902, #100271, #10576 ) ;
#56367=FACE_OUTER_BOUND ( 'NONE', #73447, .T. ) ;
#56368=CARTESIAN_POINT ( 'NONE',  ( 8.349999999999919709, 12.50000000000000000, -2.857883832488653741 ) ) ;
#56369=CARTESIAN_POINT ( 'NONE',  ( -14.39999999999998614, 2.500000000000000000, 0.3464101615137758494 ) ) ;
#56370=ORIENTED_EDGE ( 'NONE', *, *, #116910, .F. ) ;
#56371=DIRECTION ( 'NONE',  ( -0.000000000000000000, 1.000000000000000000, -0.000000000000000000 ) ) ;
#56372=CARTESIAN_POINT ( 'NONE',  ( -7.950000000000016165, 2.500000000000000000, -6.595190528383296780 ) ) ;
#56375=CARTESIAN_POINT ( 'NONE',  ( -4.600000000000025402, 2.500000000000000000, 4.430127018922196847 ) ) ;
#56376=EDGE_LOOP ( 'NONE', ( #27425, #31906 ) ) ;
#56377=ORIENTED_EDGE ( 'NONE', *, *, #120361, .T. ) ;
#56378=DIRECTION ( 'NONE',  ( 0.000000000000000000, 0.000000000000000000, 1.000000000000000000 ) ) ;
#56379=EDGE_LOOP ( 'NONE', ( #42246, #33433, #34628, #64858 ) ) ;
#56380=DIRECTION ( 'NONE',  ( -0.000000000000000000, 1.000000000000000000, -0.000000000000000000 ) ) ;
#56381=ORIENTED_EDGE ( 'NONE', *, *, #57235, .F. ) ;
#56383=EDGE_LOOP ( 'NONE', ( #118033, #109413 ) ) ;
#56384=DIRECTION ( 'NONE',  ( -0.000000000000000000, -1.000000000000000000, -0.000000000000000000 ) ) ;
#56385=VECTOR ( 'NONE', #41520, 1000.000000000000000 ) ;
#56386=DIRECTION ( 'NONE',  ( 0.000000000000000000, 0.000000000000000000, 1.000000000000000000 ) ) ;
#56387=CIRCLE ( 'NONE', #100223, 0.06509327318403745899 ) ;
#56388=CARTESIAN_POINT ( 'NONE',  ( 10.59999999999991260, 12.50000000000000000, -0.3464101615137783474 ) ) ;
#56389=DIRECTION ( 'NONE',  ( 0.000000000000000000, 0.000000000000000000, 1.000000000000000000 ) ) ;
#56390=CARTESIAN_POINT ( 'NONE',  ( 8.099999999999923261, 2.500000000000000000, -4.576537180435978236 ) ) ;
#56392=ORIENTED_EDGE ( 'NONE', *, *, #109077, .F. ) ;
#56393=EDGE_CURVE ( 'NONE', #64447, #101569, #108558, .T. ) ;
#56394=AXIS2_PLACEMENT_3D ( 'NONE', #128736, #79606, #100522 ) ;
#56395=PLANE ( 'NONE',  #28859 ) ;
#56396=CONICAL_SURFACE ( 'NONE', #89848, 0.1000000000000002554, 0.003490658503988666988 ) ;
#56397=EDGE_LOOP ( 'NONE', ( #91635, #23882 ) ) ;
#56398=EDGE_CURVE ( 'NONE', #47981, #114315, #9940, .T. ) ;
#56399=EDGE_LOOP ( 'NONE', ( #61112, #111792, #10278, #27042 ) ) ;
#56401=ORIENTED_EDGE ( 'NONE', *, *, #85061, .T. ) ;
#56402=ADVANCED_FACE ( 'NONE', ( #38556 ), #89368, .T. ) ;
#56403=CARTESIAN_POINT ( 'NONE',  ( -11.64999999999999680, 12.50000000000000000, -2.857883832488649745 ) ) ;
#56404=ORIENTED_EDGE ( 'NONE', *, *, #89620, .T. ) ;
#56405=EDGE_LOOP ( 'NONE', ( #69659, #93201, #127406, #45217 ) ) ;
#56406=AXIS2_PLACEMENT_3D ( 'NONE', #128482, #38827, #17854 ) ;
#56407=EDGE_CURVE ( 'NONE', #37781, #119461, #95622, .T. ) ;
#56408=AXIS2_PLACEMENT_3D ( 'NONE', #59709, #90409, #748 ) ;
#56409=LINE ( 'NONE', #65588, #51912 ) ;
#56410=CARTESIAN_POINT ( 'NONE',  ( 1.849999999999949685, 2.500000000000000000, 1.818653347947321475 ) ) ;
#56411=AXIS2_PLACEMENT_3D ( 'NONE', #74678, #73378, #114589 ) ;
#56412=CARTESIAN_POINT ( 'NONE',  ( -0.4000000000000339950, 2.500000000000000000, 0.6928203230275518099 ) ) ;
#56413=CARTESIAN_POINT ( 'NONE',  ( 8.749999999999920064, 2.500000000000000000, -2.757883832488654097 ) ) ;
#56414=PLANE ( 'NONE',  #94756 ) ;
#56415=VERTEX_POINT ( 'NONE', #67975 ) ;
#56416=LINE ( 'NONE', #100685, #88954 ) ;
#56417=VECTOR ( 'NONE', #16187, 1000.000000000000000 ) ;
#56418=ORIENTED_EDGE ( 'NONE', *, *, #89783, .F. ) ;
#56419=FACE_OUTER_BOUND ( 'NONE', #14253, .T. ) ;
#56420=ORIENTED_EDGE ( 'NONE', *, *, #114497, .F. ) ;
#56421=FACE_OUTER_BOUND ( 'NONE', #38778, .T. ) ;
#56422=CONICAL_SURFACE ( 'NONE', #123247, 0.1000000000000000472, 0.003490658503988666988 ) ;
#56423=VERTEX_POINT ( 'NONE', #107909 ) ;
#56424=ADVANCED_FACE ( 'NONE', ( #29367 ), #43416, .T. ) ;
#56425=ORIENTED_EDGE ( 'NONE', *, *, #67377, .T. ) ;
#56426=DIRECTION ( 'NONE',  ( 0.000000000000000000, -0.9999939076577903929, 0.003490651415223739937 ) ) ;
#56427=DIRECTION ( 'NONE',  ( 0.000000000000000000, 0.000000000000000000, -1.000000000000000000 ) ) ;
#56428=CARTESIAN_POINT ( 'NONE',  ( -2.100000000000033396, 2.500000000000000000, -3.737306695894649700 ) ) ;
#56429=DIRECTION ( 'NONE',  ( 0.000000000000000000, 0.000000000000000000, 1.000000000000000000 ) ) ;
#56431=EDGE_LOOP ( 'NONE', ( #113702, #67267, #45599, #79784 ) ) ;
#56432=DIRECTION ( 'NONE',  ( -4.274815082592931898E-19, -0.9999939076577903929, -0.003490651415223739937 ) ) ;
#56433=CARTESIAN_POINT ( 'NONE',  ( -6.650000000000015454, 2.500000000000000000, 7.188010851410848723 ) ) ;
#56434=DIRECTION ( 'NONE',  ( 0.000000000000000000, 0.000000000000000000, 1.000000000000000000 ) ) ;
#56435=DIRECTION ( 'NONE',  ( 0.000000000000000000, 1.000000000000000000, 0.000000000000000000 ) ) ;
#56436=CARTESIAN_POINT ( 'NONE',  ( 7.099999999999926814, 2.500000000000000000, -0.6928203230275541413 ) ) ;
#56437=EDGE_LOOP ( 'NONE', ( #44590, #81396, #52527 ) ) ;
#56438=ADVANCED_FACE ( 'NONE', ( #69259 ), #62187, .T. ) ;
#56440=EDGE_CURVE ( 'NONE', #16833, #113875, #5717, .T. ) ;
#56441=DIRECTION ( 'NONE',  ( -0.000000000000000000, 1.000000000000000000, -0.000000000000000000 ) ) ;
#56442=VECTOR ( 'NONE', #9065, 1000.000000000000000 ) ;
#56443=VERTEX_POINT ( 'NONE', #48346 ) ;
#56444=CARTESIAN_POINT ( 'NONE',  ( -10.45000000000000107, 2.500000000000000000, 6.595190528383296780 ) ) ;
#56445=LINE ( 'NONE', #7987, #4162 ) ;
#56446=AXIS2_PLACEMENT_3D ( 'NONE', #106359, #16664, #87987 ) ;
#56447=CIRCLE ( 'NONE', #35546, 0.06509327318403745899 ) ;
#56448=ORIENTED_EDGE ( 'NONE', *, *, #100409, .F. ) ;
#56450=CARTESIAN_POINT ( 'NONE',  ( -0.6000000000000388356, 12.50000000000000000, 4.741630453620009789 ) ) ;
#56451=FACE_OUTER_BOUND ( 'NONE', #104451, .T. ) ;
#56452=EDGE_CURVE ( 'NONE', #114810, #112120, #97673, .T. ) ;
#56453=CARTESIAN_POINT ( 'NONE',  ( 2.099999999999950351, 2.500000000000000000, -2.276824562219559311E-15 ) ) ;
#56457=CARTESIAN_POINT ( 'NONE',  ( 12.29999999999990656, 12.50000000000000000, -4.676537180435977881 ) ) ;
#56458=FACE_OUTER_BOUND ( 'NONE', #126107, .T. ) ;
#56459=ORIENTED_EDGE ( 'NONE', *, *, #117371, .F. ) ;
#56461=CARTESIAN_POINT ( 'NONE',  ( -14.14999999999998614, 2.500000000000000000, -2.065063509461099844 ) ) ;
#56462=CARTESIAN_POINT ( 'NONE',  ( 4.599999999999938360, 2.500000000000000000, -0.7928203230275542301 ) ) ;
#56463=ORIENTED_EDGE ( 'NONE', *, *, #35673, .T. ) ;
#56464=DIRECTION ( 'NONE',  ( 0.000000000000000000, 0.000000000000000000, 1.000000000000000000 ) ) ;
#56465=ORIENTED_EDGE ( 'NONE', *, *, #60048, .F. ) ;
#56466=DIRECTION ( 'NONE',  ( 0.000000000000000000, 1.000000000000000000, 0.000000000000000000 ) ) ;
#56467=CARTESIAN_POINT ( 'NONE',  ( 4.149999999999939959, 12.50000000000000000, 1.472243186433545459 ) ) ;
#56468=FACE_OUTER_BOUND ( 'NONE', #49997, .T. ) ;
#56469=ORIENTED_EDGE ( 'NONE', *, *, #68784, .T. ) ;
#56470=VECTOR ( 'NONE', #6461, 1000.000000000000000 ) ;
#56471=FACE_OUTER_BOUND ( 'NONE', #15577, .T. ) ;
#56472=CIRCLE ( 'NONE', #47, 0.06509327318403745899 ) ;
#56473=EDGE_CURVE ( 'NONE', #107710, #116926, #116539, .T. ) ;
#56474=DIRECTION ( 'NONE',  ( -0.000000000000000000, 1.000000000000000000, -0.000000000000000000 ) ) ;
#56475=EDGE_LOOP ( 'NONE', ( #62284, #8024, #10350, #35159 ) ) ;
#56476=ORIENTED_EDGE ( 'NONE', *, *, #8216, .T. ) ;
#56477=VECTOR ( 'NONE', #40559, 1000.000000000000000 ) ;
#56478=CARTESIAN_POINT ( 'NONE',  ( -1.450000000000035039, 2.500000000000000000, -2.611473670974877592 ) ) ;
#56479=EDGE_CURVE ( 'NONE', #23072, #94071, #41259, .T. ) ;
#56480=VERTEX_POINT ( 'NONE', #31940 ) ;
#56482=DIRECTION ( 'NONE',  ( -0.000000000000000000, -1.000000000000000000, -0.000000000000000000 ) ) ;
#56485=EDGE_CURVE ( 'NONE', #108498, #41959, #20827, .T. ) ;
#56486=VERTEX_POINT ( 'NONE', #40483 ) ;
#56487=EDGE_CURVE ( 'NONE', #104378, #113501, #20316, .T. ) ;
#56488=CIRCLE ( 'NONE', #60640, 0.09999999999999999167 ) ;
#56489=ADVANCED_FACE ( 'NONE', ( #71203 ), #114391, .T. ) ;
#56490=DIRECTION ( 'NONE',  ( 0.000000000000000000, 0.000000000000000000, 1.000000000000000000 ) ) ;
#56491=DIRECTION ( 'NONE',  ( -0.000000000000000000, -1.000000000000000000, -0.000000000000000000 ) ) ;
#56492=ORIENTED_EDGE ( 'NONE', *, *, #34230, .F. ) ;
#56493=AXIS2_PLACEMENT_3D ( 'NONE', #71413, #72092, #111332 ) ;
#56494=DIRECTION ( 'NONE',  ( 0.000000000000000000, 0.000000000000000000, 1.000000000000000000 ) ) ;
#56495=LINE ( 'NONE', #96412, #43071 ) ;
#56496=CONICAL_SURFACE ( 'NONE', #98350, 0.1000000000000002554, 0.003490658503988666988 ) ;
#56498=DIRECTION ( 'NONE',  ( 0.000000000000000000, 1.000000000000000000, 0.000000000000000000 ) ) ;
#56499=DIRECTION ( 'NONE',  ( 0.000000000000000000, 0.000000000000000000, 1.000000000000000000 ) ) ;
#56500=EDGE_CURVE ( 'NONE', #24462, #6208, #120670, .T. ) ;
#56501=DIRECTION ( 'NONE',  ( 0.000000000000000000, 1.000000000000000000, 0.000000000000000000 ) ) ;
#56502=LINE ( 'NONE', #57156, #96398 ) ;
#56503=EDGE_CURVE ( 'NONE', #40225, #92121, #126935, .T. ) ;
#56504=AXIS2_PLACEMENT_3D ( 'NONE', #89652, #109943, #70016 ) ;
#56505=ADVANCED_FACE ( 'NONE', ( #111786 ), #122896, .T. ) ;
#56506=ADVANCED_FACE ( 'NONE', ( #61403 ), #101962, .T. ) ;
#56507=EDGE_LOOP ( 'NONE', ( #94777, #119047, #126480, #87766 ) ) ;
#56508=EDGE_LOOP ( 'NONE', ( #25913, #5093, #1097, #74051 ) ) ;
#56509=EDGE_LOOP ( 'NONE', ( #95108, #105896, #31580, #112380 ) ) ;
#56510=EDGE_LOOP ( 'NONE', ( #128945, #120750, #50255, #41568 ) ) ;
#56511=VECTOR ( 'NONE', #74690, 1000.000000000000000 ) ;
#56512=CARTESIAN_POINT ( 'NONE',  ( -11.69999999999999574, 2.500000000000000000, 4.330127018922196314 ) ) ;
#56513=DIRECTION ( 'NONE',  ( 0.000000000000000000, 0.000000000000000000, 1.000000000000000000 ) ) ;
#56514=CARTESIAN_POINT ( 'NONE',  ( -12.29999999999999716, 12.50000000000000000, 0.2813168883297402778 ) ) ;
#56515=ORIENTED_EDGE ( 'NONE', *, *, #78521, .T. ) ;
#56516=FACE_BOUND ( 'NONE', #113186, .T. ) ;
#56517=ADVANCED_FACE ( 'NONE', ( #112435 ), #11642, .T. ) ;
#56518=DIRECTION ( 'NONE',  ( 0.000000000000000000, -0.9999939076577903929, 0.003490651415223739937 ) ) ;
#56519=CARTESIAN_POINT ( 'NONE',  ( -8.749999999999975131, 12.50000000000000000, 2.165063509461097713 ) ) ;
#56520=DIRECTION ( 'NONE',  ( 0.000000000000000000, 1.000000000000000000, 0.000000000000000000 ) ) ;
#56521=CARTESIAN_POINT ( 'NONE',  ( -5.000000000000022204, 12.50000000000000000, 3.637306695894644726 ) ) ;
#56522=CARTESIAN_POINT ( 'NONE',  ( 15.83209681635555022, -2.500000000000000000, -5.404881881984138658 ) ) ;
#56523=DIRECTION ( 'NONE',  ( 0.000000000000000000, 0.000000000000000000, 1.000000000000000000 ) ) ;
#56524=DIRECTION ( 'NONE',  ( -0.000000000000000000, -1.000000000000000000, -0.000000000000000000 ) ) ;
#56525=DIRECTION ( 'NONE',  ( -0.000000000000000000, -1.000000000000000000, -0.000000000000000000 ) ) ;
#56526=CARTESIAN_POINT ( 'NONE',  ( 2.899999999999945732, 12.50000000000000000, -4.330127018922201643 ) ) ;
#56527=DIRECTION ( 'NONE',  ( 0.000000000000000000, 0.000000000000000000, 1.000000000000000000 ) ) ;
#56528=EDGE_LOOP ( 'NONE', ( #108999, #48155 ) ) ;
#56529=ORIENTED_EDGE ( 'NONE', *, *, #72266, .F. ) ;
#56530=EDGE_LOOP ( 'NONE', ( #88753, #11486 ) ) ;
#56531=ORIENTED_EDGE ( 'NONE', *, *, #16182, .F. ) ;
#56532=DIRECTION ( 'NONE',  ( -0.000000000000000000, -1.000000000000000000, -0.000000000000000000 ) ) ;
#56533=VECTOR ( 'NONE', #50149, 1000.000000000000000 ) ;
#56534=CARTESIAN_POINT ( 'NONE',  ( 9.149999999999920419, 2.500000000000000000, 1.472243186433545459 ) ) ;
#56535=AXIS2_PLACEMENT_3D ( 'NONE', #73150, #113059, #33857 ) ;
#56536=EDGE_CURVE ( 'NONE', #94526, #44317, #124871, .T. ) ;
#56537=ORIENTED_EDGE ( 'NONE', *, *, #89485, .F. ) ;
#56539=DIRECTION ( 'NONE',  ( 0.000000000000000000, 1.000000000000000000, 0.000000000000000000 ) ) ;
#56540=CIRCLE ( 'NONE', #60676, 0.1000000000000002554 ) ;
#56541=DIRECTION ( 'NONE',  ( 0.000000000000000000, 0.000000000000000000, 1.000000000000000000 ) ) ;
#56542=DIRECTION ( 'NONE',  ( 0.000000000000000000, 0.000000000000000000, 1.000000000000000000 ) ) ;
#56543=CARTESIAN_POINT ( 'NONE',  ( -12.04999999999999716, 2.500000000000000000, -2.265063509461097802 ) ) ;
#56544=FACE_OUTER_BOUND ( 'NONE', #29392, .T. ) ;
#56545=ORIENTED_EDGE ( 'NONE', *, *, #14656, .F. ) ;
#56547=EDGE_CURVE ( 'NONE', #89132, #98092, #62692, .T. ) ;
#56548=ORIENTED_EDGE ( 'NONE', *, *, #113132, .T. ) ;
#56549=ORIENTED_EDGE ( 'NONE', *, *, #64205, .T. ) ;
#56550=ADVANCED_FACE ( 'NONE', ( #100652 ), #39314, .T. ) ;
#56551=CARTESIAN_POINT ( 'NONE',  ( -11.64999999999999680, 2.500000000000000000, 6.395190528383296602 ) ) ;
#56552=EDGE_LOOP ( 'NONE', ( #114416, #28569 ) ) ;
#56553=ORIENTED_EDGE ( 'NONE', *, *, #6504, .T. ) ;
#56554=CARTESIAN_POINT ( 'NONE',  ( -4.800000000000022915, 2.500000000000000000, -0.4464101615137783252 ) ) ;
#56555=EDGE_CURVE ( 'NONE', #2822, #74443, #10975, .T. ) ;
#56556=DIRECTION ( 'NONE',  ( -0.000000000000000000, 1.000000000000000000, -0.000000000000000000 ) ) ;
#56557=CARTESIAN_POINT ( 'NONE',  ( -4.600000000000024514, 2.500000000000000000, 3.537306695894645081 ) ) ;
#56559=DIRECTION ( 'NONE',  ( 0.000000000000000000, -0.000000000000000000, 1.000000000000000000 ) ) ;
#56560=ORIENTED_EDGE ( 'NONE', *, *, #56624, .T. ) ;
#56561=LINE ( 'NONE', #93929, #44867 ) ;
#56562=AXIS2_PLACEMENT_3D ( 'NONE', #119221, #127754, #38086 ) ;
#56563=AXIS2_PLACEMENT_3D ( 'NONE', #44997, #84905, #113071 ) ;
#56564=ORIENTED_EDGE ( 'NONE', *, *, #36495, .F. ) ;
#56565=CARTESIAN_POINT ( 'NONE',  ( 8.349999999999923261, 12.50000000000000000, 2.857883832488649301 ) ) ;
#56566=ORIENTED_EDGE ( 'NONE', *, *, #55778, .T. ) ;
#56567=DIRECTION ( 'NONE',  ( -0.000000000000000000, 1.000000000000000000, -0.000000000000000000 ) ) ;
#56568=FACE_OUTER_BOUND ( 'NONE', #77928, .T. ) ;
#56569=ORIENTED_EDGE ( 'NONE', *, *, #56126, .F. ) ;
#56570=DIRECTION ( 'NONE',  ( 0.000000000000000000, 0.000000000000000000, -1.000000000000000000 ) ) ;
#56571=LINE ( 'NONE', #37608, #22962 ) ;
#56572=ORIENTED_EDGE ( 'NONE', *, *, #83952, .T. ) ;
#56573=CONICAL_SURFACE ( 'NONE', #60797, 0.09999999999999982514, 0.003490658503988666988 ) ;
#56574=CARTESIAN_POINT ( 'NONE',  ( 0.6499999999999543920, 2.500000000000000000, 6.148780366869520897 ) ) ;
#56576=VERTEX_POINT ( 'NONE', #91491 ) ;
#56577=DIRECTION ( 'NONE',  ( 0.000000000000000000, 1.000000000000000000, 0.000000000000000000 ) ) ;
#56578=FACE_OUTER_BOUND ( 'NONE', #16622, .T. ) ;
#56580=FACE_OUTER_BOUND ( 'NONE', #1505, .T. ) ;
#56581=AXIS2_PLACEMENT_3D ( 'NONE', #68694, #60188, #28137 ) ;
#56582=ADVANCED_FACE ( 'NONE', ( #21463 ), #84891, .T. ) ;
#56583=CIRCLE ( 'NONE', #81723, 0.06509327318403745899 ) ;
#56584=CARTESIAN_POINT ( 'NONE',  ( 3.749999999999944045, 12.50000000000000000, -2.857883832488653741 ) ) ;
#56585=CARTESIAN_POINT ( 'NONE',  ( -10.80000000000000071, 2.500000000000000000, 0.09999999999999772959 ) ) ;
#56586=EDGE_CURVE ( 'NONE', #82277, #39657, #99923, .T. ) ;
#56587=AXIS2_PLACEMENT_3D ( 'NONE', #94803, #105265, #46337 ) ;
#56588=ORIENTED_EDGE ( 'NONE', *, *, #35487, .F. ) ;
#56589=PLANE ( 'NONE',  #15062 ) ;
#56590=VERTEX_POINT ( 'NONE', #105824 ) ;
#56591=AXIS2_PLACEMENT_3D ( 'NONE', #112543, #91599, #1281 ) ;
#56593=FACE_OUTER_BOUND ( 'NONE', #682, .T. ) ;
#56594=DIRECTION ( 'NONE',  ( 0.000000000000000000, 1.000000000000000000, 0.000000000000000000 ) ) ;
#56595=CARTESIAN_POINT ( 'NONE',  ( 4.599999999999938360, 12.50000000000000000, -0.6277270498435166823 ) ) ;
#56596=EDGE_CURVE ( 'NONE', #119631, #30265, #3775, .T. ) ;
#56597=DIRECTION ( 'NONE',  ( 0.000000000000000000, 1.000000000000000000, 0.000000000000000000 ) ) ;
#56598=DIRECTION ( 'NONE',  ( 0.000000000000000000, 0.000000000000000000, 1.000000000000000000 ) ) ;
#56599=ORIENTED_EDGE ( 'NONE', *, *, #61385, .F. ) ;
#56600=DIRECTION ( 'NONE',  ( 0.000000000000000000, 1.000000000000000000, 0.000000000000000000 ) ) ;
#56601=CARTESIAN_POINT ( 'NONE',  ( 2.899999999999946620, 12.50000000000000000, -0.6277270498435167934 ) ) ;
#56602=EDGE_CURVE ( 'NONE', #120278, #33691, #76851, .T. ) ;
#56603=ORIENTED_EDGE ( 'NONE', *, *, #107788, .T. ) ;
#56604=DIRECTION ( 'NONE',  ( 0.000000000000000000, -0.000000000000000000, 1.000000000000000000 ) ) ;
#56605=ORIENTED_EDGE ( 'NONE', *, *, #126109, .T. ) ;
#56606=ORIENTED_EDGE ( 'NONE', *, *, #78843, .T. ) ;
#56608=AXIS2_PLACEMENT_3D ( 'NONE', #115466, #79294, #110036 ) ;
#56609=CIRCLE ( 'NONE', #37847, 0.06509327318403745899 ) ;
#56610=CIRCLE ( 'NONE', #186, 0.1000000000000002554 ) ;
#56611=EDGE_LOOP ( 'NONE', ( #3424, #118367, #74026, #5015 ) ) ;
#56612=FACE_OUTER_BOUND ( 'NONE', #18933, .T. ) ;
#56613=DIRECTION ( 'NONE',  ( 0.000000000000000000, -0.9999939076577903929, 0.003490651415223739937 ) ) ;
#56614=FACE_OUTER_BOUND ( 'NONE', #53744, .T. ) ;
#56615=VERTEX_POINT ( 'NONE', #55436 ) ;
#56616=AXIS2_PLACEMENT_3D ( 'NONE', #57104, #78038, #25710 ) ;
#56617=FACE_BOUND ( 'NONE', #78064, .T. ) ;
#56618=DIRECTION ( 'NONE',  ( 0.000000000000000000, 0.000000000000000000, -1.000000000000000000 ) ) ;
#56619=ORIENTED_EDGE ( 'NONE', *, *, #32582, .T. ) ;
#56620=CIRCLE ( 'NONE', #92148, 0.06509327318403745899 ) ;
#56621=CARTESIAN_POINT ( 'NONE',  ( -8.750000000000012434, 2.500000000000000000, -5.802370205355744659 ) ) ;
#56622=DIRECTION ( 'NONE',  ( 0.000000000000000000, 0.000000000000000000, -1.000000000000000000 ) ) ;
#56623=ORIENTED_EDGE ( 'NONE', *, *, #63436, .F. ) ;
#56624=EDGE_CURVE ( 'NONE', #23431, #10632, #26757, .T. ) ;
#56625=EDGE_LOOP ( 'NONE', ( #21847, #49076, #115403, #79799 ) ) ;
#56626=VERTEX_POINT ( 'NONE', #105172 ) ;
#56627=CARTESIAN_POINT ( 'NONE',  ( -2.499999999999996003, 12.50000000000000000, -2.276824562219559311E-15 ) ) ;
#56628=CARTESIAN_POINT ( 'NONE',  ( 4.349999999999939249, 2.500000000000000000, 2.611473670974873151 ) ) ;
#56629=DIRECTION ( 'NONE',  ( 0.000000000000000000, 0.000000000000000000, 1.000000000000000000 ) ) ;
#56630=ADVANCED_FACE ( 'NONE', ( #66533 ), #12082, .T. ) ;
#56631=FACE_BOUND ( 'NONE', #24509, .T. ) ;
#56632=ORIENTED_EDGE ( 'NONE', *, *, #71089, .T. ) ;
#56633=EDGE_CURVE ( 'NONE', #125704, #11303, #72732, .T. ) ;
#56634=DIRECTION ( 'NONE',  ( -0.000000000000000000, 1.000000000000000000, -0.000000000000000000 ) ) ;
#56635=DIRECTION ( 'NONE',  ( 0.000000000000000000, 1.000000000000000000, 0.000000000000000000 ) ) ;
#56636=CARTESIAN_POINT ( 'NONE',  ( -17.50000000000000000, 2.500000000000000000, 1.734723475976807094E-15 ) ) ;
#56637=EDGE_CURVE ( 'NONE', #66216, #25385, #124828, .T. ) ;
#56641=ADVANCED_FACE ( 'NONE', ( #123516 ), #30892, .T. ) ;
#56642=DIRECTION ( 'NONE',  ( -0.000000000000000000, -1.000000000000000000, -0.000000000000000000 ) ) ;
#56643=DIRECTION ( 'NONE',  ( 0.000000000000000000, 0.000000000000000000, -1.000000000000000000 ) ) ;
#56644=CONICAL_SURFACE ( 'NONE', #75440, 0.09999999999999982514, 0.003490658503988666988 ) ;
#56645=CIRCLE ( 'NONE', #119358, 0.06509327318403745899 ) ;
#56648=VERTEX_POINT ( 'NONE', #95367 ) ;
#56649=ORIENTED_EDGE ( 'NONE', *, *, #25808, .T. ) ;
#56650=EDGE_LOOP ( 'NONE', ( #111093, #63795, #17089, #26949 ) ) ;
#56651=ORIENTED_EDGE ( 'NONE', *, *, #76601, .T. ) ;
#56652=CARTESIAN_POINT ( 'NONE',  ( 6.649999999999931966, 2.500000000000000000, -7.188010851410854052 ) ) ;
#56653=DIRECTION ( 'NONE',  ( 0.000000000000000000, -0.9999939076577903929, 0.003490651415223739937 ) ) ;
#56654=VERTEX_POINT ( 'NONE', #56064 ) ;
#56655=FACE_BOUND ( 'NONE', #126432, .T. ) ;
#56656=AXIS2_PLACEMENT_3D ( 'NONE', #40831, #62391, #120013 ) ;
#56657=ADVANCED_FACE ( 'NONE', ( #5670 ), #54778, .T. ) ;
#56658=DIRECTION ( 'NONE',  ( 0.000000000000000000, 0.000000000000000000, 1.000000000000000000 ) ) ;
#56659=AXIS2_PLACEMENT_3D ( 'NONE', #38742, #78655, #118553 ) ;
#56660=CARTESIAN_POINT ( 'NONE',  ( -8.350000000000013856, 2.500000000000000000, -7.288010851410849256 ) ) ;
#56661=CARTESIAN_POINT ( 'NONE',  ( 5.849999999999934808, 2.500000000000000000, -5.702370205355749455 ) ) ;
#56663=CARTESIAN_POINT ( 'NONE',  ( -1.850000000000033840, 2.500000000000000000, 6.148780366869520897 ) ) ;
#56664=ORIENTED_EDGE ( 'NONE', *, *, #42449, .T. ) ;
#56665=CARTESIAN_POINT ( 'NONE',  ( 6.899999999999926636, 12.50000000000000000, 0.2813168883297362810 ) ) ;
#56666=AXIS2_PLACEMENT_3D ( 'NONE', #56133, #96696, #7021 ) ;
#56668=VECTOR ( 'NONE', #51999, 1000.000000000000000 ) ;
#56669=EDGE_LOOP ( 'NONE', ( #14685, #101328, #123565, #22193 ) ) ;
#56670=ORIENTED_EDGE ( 'NONE', *, *, #115489, .T. ) ;
#56671=DIRECTION ( 'NONE',  ( 0.000000000000000000, 1.000000000000000000, 0.000000000000000000 ) ) ;
#56672=LINE ( 'NONE', #64576, #124991 ) ;
#56673=CARTESIAN_POINT ( 'NONE',  ( -7.950000000000012612, 2.500000000000000000, -2.265063509461101798 ) ) ;
#56674=VERTEX_POINT ( 'NONE', #44318 ) ;
#56675=FACE_OUTER_BOUND ( 'NONE', #81384, .T. ) ;
#56676=CONICAL_SURFACE ( 'NONE', #4529, 0.1000000000000002554, 0.003490658503988666988 ) ;
#56677=DIRECTION ( 'NONE',  ( 0.000000000000000000, 0.000000000000000000, -1.000000000000000000 ) ) ;
#56678=CARTESIAN_POINT ( 'NONE',  ( 4.599999999999936584, 12.50000000000000000, 4.395220292106234439 ) ) ;
#56679=AXIS2_PLACEMENT_3D ( 'NONE', #103272, #55451, #43723 ) ;
#56681=CARTESIAN_POINT ( 'NONE',  ( 0.6499999999999561684, 2.500000000000000000, -1.818653347947325916 ) ) ;
#56682=DIRECTION ( 'NONE',  ( 0.000000000000000000, -0.000000000000000000, 1.000000000000000000 ) ) ;
#56683=LINE ( 'NONE', #117533, #9875 ) ;
#56684=ORIENTED_EDGE ( 'NONE', *, *, #12323, .F. ) ;
#56685=CARTESIAN_POINT ( 'NONE',  ( -8.100000000000013856, 2.500000000000000000, -4.576537180435977348 ) ) ;
#56686=ORIENTED_EDGE ( 'NONE', *, *, #8550, .F. ) ;
#56687=EDGE_CURVE ( 'NONE', #43527, #7618, #53862, .T. ) ;
#56688=VERTEX_POINT ( 'NONE', #84237 ) ;
#56689=FACE_OUTER_BOUND ( 'NONE', #111457, .T. ) ;
#56690=FACE_OUTER_BOUND ( 'NONE', #44617, .T. ) ;
#56691=LINE ( 'NONE', #65886, #98962 ) ;
#56692=VERTEX_POINT ( 'NONE', #124174 ) ;
#56693=ORIENTED_EDGE ( 'NONE', *, *, #14144, .F. ) ;
#56694=ADVANCED_FACE ( 'NONE', ( #34529 ), #74438, .T. ) ;
#56695=CARTESIAN_POINT ( 'NONE',  ( 10.39999999999991331, 2.500000000000000000, 0.09999999999999761857 ) ) ;
#56696=CARTESIAN_POINT ( 'NONE',  ( 1.899999999999951283, 12.50000000000000000, -0.4115034346978156399 ) ) ;
#56697=AXIS2_PLACEMENT_3D ( 'NONE', #104698, #46429, #15013 ) ;
#56698=LINE ( 'NONE', #94076, #39848 ) ;
#56699=EDGE_LOOP ( 'NONE', ( #81394, #113782 ) ) ;
#56700=EDGE_LOOP ( 'NONE', ( #36895, #51802 ) ) ;
#56701=AXIS2_PLACEMENT_3D ( 'NONE', #63363, #123551, #73814 ) ;
#56702=CARTESIAN_POINT ( 'NONE',  ( 3.349999999999943689, 12.50000000000000000, 1.537336459617582918 ) ) ;
#56703=VERTEX_POINT ( 'NONE', #35171 ) ;
#56704=LINE ( 'NONE', #5040, #79222 ) ;
#56705=AXIS2_PLACEMENT_3D ( 'NONE', #96214, #46474, #76592 ) ;
#56706=DIRECTION ( 'NONE',  ( 0.000000000000000000, 1.000000000000000000, 0.000000000000000000 ) ) ;
#56707=ORIENTED_EDGE ( 'NONE', *, *, #105380, .T. ) ;
#56708=CARTESIAN_POINT ( 'NONE',  ( -7.900000000000014566, 2.500000000000000000, -0.6928203230275541413 ) ) ;
#56709=DIRECTION ( 'NONE',  ( 0.000000000000000000, -0.000000000000000000, 1.000000000000000000 ) ) ;
#56710=DIRECTION ( 'NONE',  ( 0.000000000000000000, 1.000000000000000000, 0.000000000000000000 ) ) ;
#56711=CIRCLE ( 'NONE', #121471, 0.06509327318403745899 ) ;
#56712=DIRECTION ( 'NONE',  ( 0.000000000000000000, 1.000000000000000000, 0.000000000000000000 ) ) ;
#56713=EDGE_LOOP ( 'NONE', ( #77258, #103193, #40739, #120513 ) ) ;
#56714=LINE ( 'NONE', #96645, #61354 ) ;
#56715=FACE_OUTER_BOUND ( 'NONE', #122413, .T. ) ;
#56716=VERTEX_POINT ( 'NONE', #68467 ) ;
#56717=ORIENTED_EDGE ( 'NONE', *, *, #7040, .T. ) ;
#56719=CARTESIAN_POINT ( 'NONE',  ( 9.349999999999919709, 12.50000000000000000, 1.818653347947321475 ) ) ;
#56720=FACE_OUTER_BOUND ( 'NONE', #89989, .T. ) ;
#56721=DIRECTION ( 'NONE',  ( -0.000000000000000000, -1.000000000000000000, -0.000000000000000000 ) ) ;
#56722=DIRECTION ( 'NONE',  ( 0.000000000000000000, -0.000000000000000000, 1.000000000000000000 ) ) ;
#56723=DIRECTION ( 'NONE',  ( -0.000000000000000000, -1.000000000000000000, -0.000000000000000000 ) ) ;
#56724=EDGE_CURVE ( 'NONE', #49230, #114968, #118695, .T. ) ;
#56725=DIRECTION ( 'NONE',  ( 0.000000000000000000, 1.000000000000000000, 0.000000000000000000 ) ) ;
#56726=FACE_OUTER_BOUND ( 'NONE', #42472, .T. ) ;
#56727=CARTESIAN_POINT ( 'NONE',  ( -9.550000000000006040, 2.500000000000000000, -2.065063509461102065 ) ) ;
#56728=DIRECTION ( 'NONE',  ( 0.000000000000000000, 0.000000000000000000, 1.000000000000000000 ) ) ;
#56729=CONICAL_SURFACE ( 'NONE', #94404, 0.09999999999999982514, 0.003490658503988666988 ) ;
#56730=EDGE_CURVE ( 'NONE', #125196, #58516, #127027, .T. ) ;
#56731=EDGE_LOOP ( 'NONE', ( #49561, #99073, #124685, #34815 ) ) ;
#56732=CONICAL_SURFACE ( 'NONE', #35839, 0.09999999999999982514, 0.003490658503988666988 ) ;
#56733=EDGE_LOOP ( 'NONE', ( #102897, #74228, #125797, #105288 ) ) ;
#56734=CARTESIAN_POINT ( 'NONE',  ( 1.049999999999952971, 2.500000000000000000, 6.248780366869521430 ) ) ;
#56735=EDGE_CURVE ( 'NONE', #79023, #118813, #104032, .T. ) ;
#56736=ORIENTED_EDGE ( 'NONE', *, *, #92554, .T. ) ;
#56737=CARTESIAN_POINT ( 'NONE',  ( 8.549999999999918998, 2.500000000000000000, 6.841600689897072485 ) ) ;
#56738=ADVANCED_FACE ( 'NONE', ( #39051 ), #81059, .T. ) ;
#56739=DIRECTION ( 'NONE',  ( 0.000000000000000000, 0.000000000000000000, 1.000000000000000000 ) ) ;
#56741=AXIS2_PLACEMENT_3D ( 'NONE', #108588, #118401, #57563 ) ;
#56742=VERTEX_POINT ( 'NONE', #59331 ) ;
#56743=DIRECTION ( 'NONE',  ( -4.274815082592931898E-19, -0.9999939076577903929, -0.003490651415223739937 ) ) ;
#56744=AXIS2_PLACEMENT_3D ( 'NONE', #11528, #12160, #100552 ) ;
#56745=EDGE_CURVE ( 'NONE', #109816, #26449, #33041, .T. ) ;
#56746=DIRECTION ( 'NONE',  ( -0.000000000000000000, -1.000000000000000000, -0.000000000000000000 ) ) ;
#56747=DIRECTION ( 'NONE',  ( 0.000000000000000000, 0.000000000000000000, 1.000000000000000000 ) ) ;
#56748=VERTEX_POINT ( 'NONE', #78317 ) ;
#56749=EDGE_CURVE ( 'NONE', #116833, #49349, #49505, .T. ) ;
#56750=DIRECTION ( 'NONE',  ( 0.000000000000000000, 0.000000000000000000, -1.000000000000000000 ) ) ;
#56751=CIRCLE ( 'NONE', #17025, 0.06509327318403745899 ) ;
#56752=ORIENTED_EDGE ( 'NONE', *, *, #112971, .T. ) ;
#56753=AXIS2_PLACEMENT_3D ( 'NONE', #4800, #45402, #44755 ) ;
#56754=EDGE_LOOP ( 'NONE', ( #53971, #116149 ) ) ;
#56755=VERTEX_POINT ( 'NONE', #18730 ) ;
#56756=CIRCLE ( 'NONE', #48383, 0.1000000000000002554 ) ;
#56757=ORIENTED_EDGE ( 'NONE', *, *, #84103, .T. ) ;
#56758=DIRECTION ( 'NONE',  ( 0.000000000000000000, -0.000000000000000000, 1.000000000000000000 ) ) ;
#56759=CIRCLE ( 'NONE', #35865, 0.06509327318403743123 ) ;
#56760=CARTESIAN_POINT ( 'NONE',  ( 21.34481565588170682, 0.7053969147713127219, 2.184679923000720336 ) ) ;
#56761=DIRECTION ( 'NONE',  ( -0.000000000000000000, -1.000000000000000000, -0.000000000000000000 ) ) ;
#56762=LINE ( 'NONE', #96697, #64502 ) ;
#56763=ORIENTED_EDGE ( 'NONE', *, *, #12195, .T. ) ;
#56764=EDGE_CURVE ( 'NONE', #97882, #101949, #41356, .T. ) ;
#56765=AXIS2_PLACEMENT_3D ( 'NONE', #9347, #47995, #49295 ) ;
#56766=AXIS2_PLACEMENT_3D ( 'NONE', #2306, #42263, #74938 ) ;
#56767=FACE_OUTER_BOUND ( 'NONE', #40160, .T. ) ;
#56768=ORIENTED_EDGE ( 'NONE', *, *, #21666, .T. ) ;
#56769=CARTESIAN_POINT ( 'NONE',  ( -3.550000000000030909, 2.500000000000000000, -6.941600689897078347 ) ) ;
#56770=DIRECTION ( 'NONE',  ( -4.274815082592931898E-19, -0.9999939076577903929, -0.003490651415223739937 ) ) ;
#56772=DIRECTION ( 'NONE',  ( 0.000000000000000000, -0.000000000000000000, 1.000000000000000000 ) ) ;
#56773=ORIENTED_EDGE ( 'NONE', *, *, #53163, .F. ) ;
#56774=EDGE_CURVE ( 'NONE', #111073, #27457, #49767, .T. ) ;
#56775=ORIENTED_EDGE ( 'NONE', *, *, #22584, .F. ) ;
#56776=ORIENTED_EDGE ( 'NONE', *, *, #83692, .T. ) ;
#56777=ORIENTED_EDGE ( 'NONE', *, *, #76762, .T. ) ;
#56778=FACE_OUTER_BOUND ( 'NONE', #87081, .T. ) ;
#56779=CARTESIAN_POINT ( 'NONE',  ( -11.64999999999999680, 12.50000000000000000, 7.253104124594885960 ) ) ;
#56780=DIRECTION ( 'NONE',  ( 0.000000000000000000, 0.000000000000000000, 1.000000000000000000 ) ) ;
#56781=FACE_BOUND ( 'NONE', #51010, .T. ) ;
#56783=CARTESIAN_POINT ( 'NONE',  ( -7.100000000000013856, 12.50000000000000000, 5.088040615133786027 ) ) ;
#56784=ADVANCED_FACE ( 'NONE', ( #39694 ), #112454, .T. ) ;
#56785=DIRECTION ( 'NONE',  ( 0.000000000000000000, 0.000000000000000000, 1.000000000000000000 ) ) ;
#56786=DIRECTION ( 'NONE',  ( 0.000000000000000000, -0.9999939076577903929, 0.003490651415223739937 ) ) ;
#56787=VECTOR ( 'NONE', #58273, 1000.000000000000000 ) ;
#56789=EDGE_CURVE ( 'NONE', #106091, #110912, #6946, .T. ) ;
#56791=CIRCLE ( 'NONE', #106976, 0.06509327318403745899 ) ;
#56794=DIRECTION ( 'NONE',  ( 0.000000000000000000, 0.000000000000000000, 1.000000000000000000 ) ) ;
#56795=EDGE_CURVE ( 'NONE', #121408, #104331, #35091, .T. ) ;
#56796=DIRECTION ( 'NONE',  ( 0.000000000000000000, -0.9999939076577903929, 0.003490651415223739937 ) ) ;
#56797=CONICAL_SURFACE ( 'NONE', #372, 0.09999999999999982514, 0.003490658503988666988 ) ;
#56798=EDGE_CURVE ( 'NONE', #111188, #93106, #74793, .T. ) ;
#56799=ORIENTED_EDGE ( 'NONE', *, *, #24608, .T. ) ;
#56800=ORIENTED_EDGE ( 'NONE', *, *, #36268, .T. ) ;
#56801=ORIENTED_EDGE ( 'NONE', *, *, #24924, .T. ) ;
#56802=ORIENTED_EDGE ( 'NONE', *, *, #77026, .T. ) ;
#56803=AXIS2_PLACEMENT_3D ( 'NONE', #69083, #38363, #109001 ) ;
#56804=CIRCLE ( 'NONE', #65222, 0.1000000000000000472 ) ;
#56805=DIRECTION ( 'NONE',  ( 0.000000000000000000, 0.000000000000000000, 1.000000000000000000 ) ) ;
#56806=FACE_BOUND ( 'NONE', #54568, .T. ) ;
#56807=DIRECTION ( 'NONE',  ( -0.000000000000000000, 1.000000000000000000, -0.000000000000000000 ) ) ;
#56808=EDGE_CURVE ( 'NONE', #43342, #42494, #91511, .T. ) ;
#56809=CIRCLE ( 'NONE', #113265, 0.09999999999999982514 ) ;
#56810=DIRECTION ( 'NONE',  ( 0.000000000000000000, 0.000000000000000000, 1.000000000000000000 ) ) ;
#56811=EDGE_CURVE ( 'NONE', #124471, #40728, #51812, .T. ) ;
#56812=VERTEX_POINT ( 'NONE', #67152 ) ;
#56813=DIRECTION ( 'NONE',  ( 0.000000000000000000, 0.000000000000000000, 1.000000000000000000 ) ) ;
#56815=EDGE_LOOP ( 'NONE', ( #88509, #52403 ) ) ;
#56816=DIRECTION ( 'NONE',  ( -0.000000000000000000, 1.000000000000000000, -0.000000000000000000 ) ) ;
#56817=CARTESIAN_POINT ( 'NONE',  ( -9.150000000000009237, 2.500000000000000000, 2.957883832488649389 ) ) ;
#56818=ORIENTED_EDGE ( 'NONE', *, *, #48529, .F. ) ;
#56819=CARTESIAN_POINT ( 'NONE',  ( 6.049999999999934097, 12.50000000000000000, -6.148780366869526226 ) ) ;
#56820=LINE ( 'NONE', #105949, #126952 ) ;
#56821=CIRCLE ( 'NONE', #10853, 0.1000000000000000472 ) ;
#56822=AXIS2_PLACEMENT_3D ( 'NONE', #13267, #81395, #112781 ) ;
#56823=ORIENTED_EDGE ( 'NONE', *, *, #99245, .F. ) ;
#56824=CARTESIAN_POINT ( 'NONE',  ( 3.549999999999942979, 2.500000000000000000, 1.718653347947321386 ) ) ;
#56825=DIRECTION ( 'NONE',  ( 0.000000000000000000, -0.000000000000000000, 1.000000000000000000 ) ) ;
#56826=VERTEX_POINT ( 'NONE', #47560 ) ;
#56827=DIRECTION ( 'NONE',  ( 0.000000000000000000, -0.000000000000000000, 1.000000000000000000 ) ) ;
#56828=ORIENTED_EDGE ( 'NONE', *, *, #84726, .F. ) ;
#56829=EDGE_LOOP ( 'NONE', ( #60184, #37566 ) ) ;
#56830=DIRECTION ( 'NONE',  ( 0.000000000000000000, 0.000000000000000000, -1.000000000000000000 ) ) ;
#56831=CIRCLE ( 'NONE', #4592, 0.1000000000000002554 ) ;
#56832=VERTEX_POINT ( 'NONE', #107097 ) ;
#56833=DIRECTION ( 'NONE',  ( -4.274815082592931898E-19, -0.9999939076577903929, -0.003490651415223739937 ) ) ;
#56834=AXIS2_PLACEMENT_3D ( 'NONE', #11489, #111627, #121433 ) ;
#56835=FACE_OUTER_BOUND ( 'NONE', #25297, .T. ) ;
#56836=AXIS2_PLACEMENT_3D ( 'NONE', #70766, #18443, #49856 ) ;
#56837=EDGE_LOOP ( 'NONE', ( #116120, #87022, #104497, #86046 ) ) ;
#56838=CONICAL_SURFACE ( 'NONE', #81999, 0.1000000000000002554, 0.003490658503988666988 ) ;
#56839=EDGE_CURVE ( 'NONE', #72411, #82981, #22579, .T. ) ;
#56840=CARTESIAN_POINT ( 'NONE',  ( 1.849999999999949019, 12.50000000000000000, 6.841600689897072485 ) ) ;
#56841=VERTEX_POINT ( 'NONE', #18078 ) ;
#56842=CARTESIAN_POINT ( 'NONE',  ( -3.350000000000028955, 12.50000000000000000, 5.802370205355744659 ) ) ;
#56843=CARTESIAN_POINT ( 'NONE',  ( 3.549999999999943867, 2.500000000000000000, -1.818653347947326138 ) ) ;
#56844=DIRECTION ( 'NONE',  ( -0.000000000000000000, -1.000000000000000000, -0.000000000000000000 ) ) ;
#56845=CARTESIAN_POINT ( 'NONE',  ( -9.999999999999971578, 12.50000000000000000, -4.330127018922197202 ) ) ;
#56846=DIRECTION ( 'NONE',  ( 0.000000000000000000, 1.000000000000000000, 0.000000000000000000 ) ) ;
#56847=ORIENTED_EDGE ( 'NONE', *, *, #117105, .F. ) ;
#56848=AXIS2_PLACEMENT_3D ( 'NONE', #73396, #94319, #113324 ) ;
#56850=ORIENTED_EDGE ( 'NONE', *, *, #24840, .F. ) ;
#56851=DIRECTION ( 'NONE',  ( 0.000000000000000000, 0.000000000000000000, 1.000000000000000000 ) ) ;
#56852=CARTESIAN_POINT ( 'NONE',  ( -8.950000000000004619, 2.500000000000000000, 6.148780366869520897 ) ) ;
#56853=AXIS2_PLACEMENT_3D ( 'NONE', #120580, #100924, #90456 ) ;
#56854=VECTOR ( 'NONE', #83311, 1000.000000000000000 ) ;
#56855=CIRCLE ( 'NONE', #67308, 0.06509327318403745899 ) ;
#56856=DIRECTION ( 'NONE',  ( 0.000000000000000000, 0.000000000000000000, 1.000000000000000000 ) ) ;
#56857=ORIENTED_EDGE ( 'NONE', *, *, #100470, .F. ) ;
#56858=ORIENTED_EDGE ( 'NONE', *, *, #53226, .T. ) ;
#56859=ORIENTED_EDGE ( 'NONE', *, *, #18128, .T. ) ;
#56860=LINE ( 'NONE', #126923, #25016 ) ;
#56861=CONICAL_SURFACE ( 'NONE', #98729, 0.1000000000000002554, 0.003490658503988666988 ) ;
#56863=CARTESIAN_POINT ( 'NONE',  ( 2.499999999999981792, 12.50000000000000000, 4.330127018922196314 ) ) ;
#56865=CARTESIAN_POINT ( 'NONE',  ( -5.650000000000023448, 2.500000000000000000, -6.841600689897078702 ) ) ;
#56866=AXIS2_PLACEMENT_3D ( 'NONE', #17707, #49138, #57654 ) ;
#56867=DIRECTION ( 'NONE',  ( 0.000000000000000000, 1.000000000000000000, 0.000000000000000000 ) ) ;
#56868=CARTESIAN_POINT ( 'NONE',  ( 0.8499999999999553468, 2.500000000000000000, -2.165063509461101710 ) ) ;
#56869=LINE ( 'NONE', #47089, #26243 ) ;
#56870=DIRECTION ( 'NONE',  ( 0.000000000000000000, 0.000000000000000000, 1.000000000000000000 ) ) ;
#56871=CARTESIAN_POINT ( 'NONE',  ( 10.84999999999991260, 2.500000000000000000, -1.372243186433550033 ) ) ;
#56872=ORIENTED_EDGE ( 'NONE', *, *, #1544, .F. ) ;
#56873=FACE_OUTER_BOUND ( 'NONE', #29838, .T. ) ;
#56874=ORIENTED_EDGE ( 'NONE', *, *, #104266, .F. ) ;
#56875=EDGE_LOOP ( 'NONE', ( #116791, #33058, #74168, #33454 ) ) ;
#56876=DIRECTION ( 'NONE',  ( 0.000000000000000000, 0.000000000000000000, 1.000000000000000000 ) ) ;
#56877=DIRECTION ( 'NONE',  ( 0.000000000000000000, -0.9999939076577903929, 0.003490651415223739937 ) ) ;
#56878=DIRECTION ( 'NONE',  ( 0.000000000000000000, 0.000000000000000000, -1.000000000000000000 ) ) ;
#56879=LINE ( 'NONE', #4547, #94415 ) ;
#56880=CARTESIAN_POINT ( 'NONE',  ( -8.100000000000010303, 12.50000000000000000, 3.918623584224383727 ) ) ;
#56881=CARTESIAN_POINT ( 'NONE',  ( -10.45000000000000462, 12.50000000000000000, -6.495190528383298911 ) ) ;
#56882=AXIS2_PLACEMENT_3D ( 'NONE', #112370, #43641, #123456 ) ;
#56883=CARTESIAN_POINT ( 'NONE',  ( -8.750000000000010658, 2.500000000000000000, -1.472243186433550122 ) ) ;
#56884=ORIENTED_EDGE ( 'NONE', *, *, #13971, .F. ) ;
#56885=CARTESIAN_POINT ( 'NONE',  ( 8.549999999999924327, 12.50000000000000000, -6.841600689897077814 ) ) ;
#56886=VECTOR ( 'NONE', #114, 1000.000000000000000 ) ;
#56887=AXIS2_PLACEMENT_3D ( 'NONE', #11822, #72055, #111294 ) ;
#56888=DIRECTION ( 'NONE',  ( 0.000000000000000000, 0.000000000000000000, 1.000000000000000000 ) ) ;
#56889=ORIENTED_EDGE ( 'NONE', *, *, #112739, .T. ) ;
#56890=EDGE_CURVE ( 'NONE', #33973, #110810, #123755, .T. ) ;
#56891=ORIENTED_EDGE ( 'NONE', *, *, #33906, .T. ) ;
#56892=CONICAL_SURFACE ( 'NONE', #10911, 0.1000000000000002554, 0.003490658503988666988 ) ;
#56893=VERTEX_POINT ( 'NONE', #112282 ) ;
#56894=CONICAL_SURFACE ( 'NONE', #65221, 0.1000000000000002554, 0.003490658503988666988 ) ;
#56895=EDGE_CURVE ( 'NONE', #42690, #6759, #125801, .T. ) ;
#56896=AXIS2_PLACEMENT_3D ( 'NONE', #30674, #68635, #40495 ) ;
#56897=EDGE_CURVE ( 'NONE', #13178, #22580, #109066, .T. ) ;
#56898=VERTEX_POINT ( 'NONE', #21975 ) ;
#56899=EDGE_LOOP ( 'NONE', ( #62118, #96849 ) ) ;
#56900=EDGE_CURVE ( 'NONE', #29791, #76636, #81525, .T. ) ;
#56901=DIRECTION ( 'NONE',  ( -4.274815082592931898E-19, -0.9999939076577903929, -0.003490651415223739937 ) ) ;
#56902=CARTESIAN_POINT ( 'NONE',  ( 11.84999999999990727, 2.500000000000000000, 6.148780366869520009 ) ) ;
#56903=CONICAL_SURFACE ( 'NONE', #111283, 0.1000000000000000056, 0.003490658503988666988 ) ;
#56904=EDGE_LOOP ( 'NONE', ( #36985, #98686 ) ) ;
#56905=CARTESIAN_POINT ( 'NONE',  ( -13.29999999999999005, 12.50000000000000000, -4.330127018922198978 ) ) ;
#56906=DIRECTION ( 'NONE',  ( 0.000000000000000000, 0.000000000000000000, -1.000000000000000000 ) ) ;
#56907=ADVANCED_FACE ( 'NONE', ( #31152 ), #90695, .T. ) ;
#56908=CARTESIAN_POINT ( 'NONE',  ( 3.949999999999938893, 2.500000000000000000, 6.048780366869520364 ) ) ;
#56909=ADVANCED_FACE ( 'NONE', ( #1022 ), #2964, .T. ) ;
#56910=ORIENTED_EDGE ( 'NONE', *, *, #84789, .F. ) ;
#56911=ADVANCED_FACE ( 'NONE', ( #30513 ), #110958, .T. ) ;
#56912=FACE_OUTER_BOUND ( 'NONE', #13779, .T. ) ;
#56913=DIRECTION ( 'NONE',  ( -0.000000000000000000, -1.000000000000000000, -0.000000000000000000 ) ) ;
#56914=EDGE_LOOP ( 'NONE', ( #100087, #96302 ) ) ;
#56915=ORIENTED_EDGE ( 'NONE', *, *, #121216, .T. ) ;
#56916=ORIENTED_EDGE ( 'NONE', *, *, #43954, .F. ) ;
#56917=LINE ( 'NONE', #128937, #50952 ) ;
#56918=AXIS2_PLACEMENT_3D ( 'NONE', #63211, #103136, #122781 ) ;
#56919=CARTESIAN_POINT ( 'NONE',  ( 11.69999999999990870, 2.500000000000000000, -4.330127018922201643 ) ) ;
#56920=CONICAL_SURFACE ( 'NONE', #65544, 0.1000000000000002554, 0.003490658503988666988 ) ;
#56921=ORIENTED_EDGE ( 'NONE', *, *, #73083, .T. ) ;
#56922=CARTESIAN_POINT ( 'NONE',  ( 8.299999999999922551, 12.50000000000000000, 4.265033745738159077 ) ) ;
#56923=DIRECTION ( 'NONE',  ( 0.000000000000000000, 0.000000000000000000, 1.000000000000000000 ) ) ;
#56924=DIRECTION ( 'NONE',  ( -0.000000000000000000, -1.000000000000000000, -0.000000000000000000 ) ) ;
#56925=CARTESIAN_POINT ( 'NONE',  ( -13.34999999999999076, 2.500000000000000000, -2.165063509461099489 ) ) ;
#56926=CIRCLE ( 'NONE', #44432, 0.06509327318403745899 ) ;
#56928=AXIS2_PLACEMENT_3D ( 'NONE', #62347, #104812, #123814 ) ;
#56929=ORIENTED_EDGE ( 'NONE', *, *, #82081, .F. ) ;
#56930=DIRECTION ( 'NONE',  ( -0.000000000000000000, 1.000000000000000000, -0.000000000000000000 ) ) ;
#56931=CIRCLE ( 'NONE', #73670, 0.06509327318403741736 ) ;
#56932=VERTEX_POINT ( 'NONE', #101812 ) ;
#56933=ORIENTED_EDGE ( 'NONE', *, *, #81243, .T. ) ;
#56934=ORIENTED_EDGE ( 'NONE', *, *, #35540, .T. ) ;
#56936=FACE_BOUND ( 'NONE', #76034, .T. ) ;
#56937=LINE ( 'NONE', #65486, #40905 ) ;
#56938=AXIS2_PLACEMENT_3D ( 'NONE', #113152, #92214, #13653 ) ;
#56939=PLANE ( 'NONE',  #92469 ) ;
#56940=VECTOR ( 'NONE', #96905, 1000.000000000000000 ) ;
#56941=DIRECTION ( 'NONE',  ( 0.000000000000000000, 0.000000000000000000, -1.000000000000000000 ) ) ;
#56944=AXIS2_PLACEMENT_3D ( 'NONE', #32097, #111931, #42565 ) ;
#56945=ADVANCED_FACE ( 'NONE', ( #42248 ), #127962, .T. ) ;
#56946=ORIENTED_EDGE ( 'NONE', *, *, #25474, .T. ) ;
#56947=EDGE_CURVE ( 'NONE', #73847, #33436, #104874, .T. ) ;
#56950=DIRECTION ( 'NONE',  ( 0.000000000000000000, -0.000000000000000000, 1.000000000000000000 ) ) ;
#56951=AXIS2_PLACEMENT_3D ( 'NONE', #6405, #57485, #116380 ) ;
#56952=EDGE_CURVE ( 'NONE', #129059, #2089, #100758, .T. ) ;
#56953=DIRECTION ( 'NONE',  ( -0.000000000000000000, -1.000000000000000000, -0.000000000000000000 ) ) ;
#56954=ORIENTED_EDGE ( 'NONE', *, *, #50753, .F. ) ;
#56955=DIRECTION ( 'NONE',  ( 0.000000000000000000, -0.000000000000000000, 1.000000000000000000 ) ) ;
#56957=CONICAL_SURFACE ( 'NONE', #4627, 0.09999999999999982514, 0.003490658503988666988 ) ;
#56958=ADVANCED_FACE ( 'NONE', ( #80888 ), #14969, .T. ) ;
#56959=ADVANCED_FACE ( 'NONE', ( #52072 ), #19188, .T. ) ;
#56960=EDGE_LOOP ( 'NONE', ( #107975, #120594 ) ) ;
#56961=DIRECTION ( 'NONE',  ( -0.000000000000000000, 1.000000000000000000, -0.000000000000000000 ) ) ;
#56962=EDGE_CURVE ( 'NONE', #18946, #50137, #91983, .T. ) ;
#56963=CARTESIAN_POINT ( 'NONE',  ( -10.20000000000000284, 2.500000000000000000, 3.983716857408420964 ) ) ;
#56964=FACE_BOUND ( 'NONE', #39954, .T. ) ;
#56965=DIRECTION ( 'NONE',  ( 0.000000000000000000, 0.000000000000000000, -1.000000000000000000 ) ) ;
#56966=EDGE_CURVE ( 'NONE', #48345, #101934, #51436, .T. ) ;
#56967=EDGE_CURVE ( 'NONE', #116425, #41491, #48454, .T. ) ;
#56968=ORIENTED_EDGE ( 'NONE', *, *, #121219, .F. ) ;
#56969=FACE_OUTER_BOUND ( 'NONE', #14278, .T. ) ;
#56970=ORIENTED_EDGE ( 'NONE', *, *, #72212, .F. ) ;
#56971=ORIENTED_EDGE ( 'NONE', *, *, #87871, .F. ) ;
#56972=CARTESIAN_POINT ( 'NONE',  ( 17.19804440726973382, 0.4677972980984265172, -5.492654682185373893 ) ) ;
#56973=VECTOR ( 'NONE', #87814, 1000.000000000000000 ) ;
#56975=ADVANCED_FACE ( 'NONE', ( #71699 ), #358, .T. ) ;
#56976=ORIENTED_EDGE ( 'NONE', *, *, #109463, .F. ) ;
#56978=DIRECTION ( 'NONE',  ( 0.000000000000000000, 0.000000000000000000, 1.000000000000000000 ) ) ;
#56979=CIRCLE ( 'NONE', #15104, 0.06509327318403745899 ) ;
#56980=DIRECTION ( 'NONE',  ( 0.000000000000000000, 1.000000000000000000, 0.000000000000000000 ) ) ;
#56981=CIRCLE ( 'NONE', #69505, 0.1000000000000000472 ) ;
#56982=CIRCLE ( 'NONE', #27749, 0.06509327318403745899 ) ;
#56983=DIRECTION ( 'NONE',  ( 0.000000000000000000, 0.000000000000000000, 1.000000000000000000 ) ) ;
#56984=AXIS2_PLACEMENT_3D ( 'NONE', #45167, #63515, #15015 ) ;
#56985=CIRCLE ( 'NONE', #82041, 0.1000000000000002554 ) ;
#56986=VERTEX_POINT ( 'NONE', #53357 ) ;
#56987=CIRCLE ( 'NONE', #123899, 0.1000000000000002554 ) ;
#56988=DIRECTION ( 'NONE',  ( 0.000000000000000000, 0.000000000000000000, 1.000000000000000000 ) ) ;
#56989=DIRECTION ( 'NONE',  ( 0.000000000000000000, 0.000000000000000000, 1.000000000000000000 ) ) ;
#56990=DIRECTION ( 'NONE',  ( 0.000000000000000000, 0.000000000000000000, 1.000000000000000000 ) ) ;
#56991=VECTOR ( 'NONE', #69253, 1000.000000000000000 ) ;
#56992=CARTESIAN_POINT ( 'NONE',  ( 12.89999999999990266, 12.50000000000000000, -3.637306695894650055 ) ) ;
#56993=CIRCLE ( 'NONE', #23567, 0.06509327318403745899 ) ;
#56994=VERTEX_POINT ( 'NONE', #105008 ) ;
#56995=CARTESIAN_POINT ( 'NONE',  ( 8.549999999999922551, 12.50000000000000000, 2.511473670974873507 ) ) ;
#56996=VECTOR ( 'NONE', #119997, 1000.000000000000000 ) ;
#56997=VERTEX_POINT ( 'NONE', #46106 ) ;
#56998=PLANE ( 'NONE',  #3305 ) ;
#56999=CARTESIAN_POINT ( 'NONE',  ( -5.850000000000021849, 2.500000000000000000, -2.757883832488654097 ) ) ;
#57000=AXIS2_PLACEMENT_3D ( 'NONE', #62574, #121460, #93311 ) ;
#57001=EDGE_LOOP ( 'NONE', ( #12076, #34516 ) ) ;
#57002=FACE_OUTER_BOUND ( 'NONE', #109895, .T. ) ;
#57003=DIRECTION ( 'NONE',  ( 0.000000000000000000, -0.9999939076577903929, 0.003490651415223739937 ) ) ;
#57004=CARTESIAN_POINT ( 'NONE',  ( -11.25000000000000000, 2.500000000000000000, -2.957883832488649833 ) ) ;
#57005=CARTESIAN_POINT ( 'NONE',  ( -5.400000000000020783, 12.50000000000000000, 0.6928203230275494784 ) ) ;
#57006=EDGE_LOOP ( 'NONE', ( #78732, #8442, #114999, #124340 ) ) ;
#57007=CARTESIAN_POINT ( 'NONE',  ( -5.400000000000019895, 2.500000000000000000, -0.1000000000000022815 ) ) ;
#57008=CARTESIAN_POINT ( 'NONE',  ( 6.249999999999928946, 2.500000000000000000, 2.757883832488649656 ) ) ;
#57009=DIRECTION ( 'NONE',  ( -4.274815082592931898E-19, -0.9999939076577903929, -0.003490651415223739937 ) ) ;
#57010=PLANE ( 'NONE',  #73595 ) ;
#57011=DIRECTION ( 'NONE',  ( 0.000000000000000000, 0.000000000000000000, -1.000000000000000000 ) ) ;
#57012=CIRCLE ( 'NONE', #8896, 0.06509327318403745899 ) ;
#57013=ORIENTED_EDGE ( 'NONE', *, *, #7006, .F. ) ;
#57014=ADVANCED_FACE ( 'NONE', ( #34372 ), #31737, .T. ) ;
#57015=ORIENTED_EDGE ( 'NONE', *, *, #118114, .F. ) ;
#57016=DIRECTION ( 'NONE',  ( 0.000000000000000000, 1.000000000000000000, 0.000000000000000000 ) ) ;
#57017=ORIENTED_EDGE ( 'NONE', *, *, #20753, .T. ) ;
#57018=DIRECTION ( 'NONE',  ( -0.000000000000000000, -1.000000000000000000, -0.000000000000000000 ) ) ;
#57019=ORIENTED_EDGE ( 'NONE', *, *, #73835, .T. ) ;
#57020=ORIENTED_EDGE ( 'NONE', *, *, #75814, .T. ) ;
#57021=ORIENTED_EDGE ( 'NONE', *, *, #77336, .F. ) ;
#57023=CIRCLE ( 'NONE', #100934, 0.06509327318403745899 ) ;
#57024=CIRCLE ( 'NONE', #100935, 0.1000000000000002554 ) ;
#57025=PLANE ( 'NONE',  #94465 ) ;
#57026=VECTOR ( 'NONE', #75997, 1000.000000000000000 ) ;
#57027=PLANE ( 'NONE',  #94949 ) ;
#57029=DIRECTION ( 'NONE',  ( 0.000000000000000000, 0.000000000000000000, 1.000000000000000000 ) ) ;
#57030=CARTESIAN_POINT ( 'NONE',  ( -8.750000000000007105, 12.50000000000000000, 7.253104124594885960 ) ) ;
#57031=LINE ( 'NONE', #87140, #99883 ) ;
#57032=ORIENTED_EDGE ( 'NONE', *, *, #49298, .T. ) ;
#57033=CIRCLE ( 'NONE', #103007, 0.1000000000000000472 ) ;
#57034=DIRECTION ( 'NONE',  ( 0.000000000000000000, -0.000000000000000000, 1.000000000000000000 ) ) ;
#57036=AXIS2_PLACEMENT_3D ( 'NONE', #26283, #106753, #38023 ) ;
#57037=ORIENTED_EDGE ( 'NONE', *, *, #37887, .T. ) ;
#57038=ORIENTED_EDGE ( 'NONE', *, *, #42782, .F. ) ;
#57039=AXIS2_PLACEMENT_3D ( 'NONE', #116014, #26364, #19081 ) ;
#57040=VERTEX_POINT ( 'NONE', #93921 ) ;
#57041=CARTESIAN_POINT ( 'NONE',  ( 0.3999999999999628852, 2.500000000000000000, -0.7928203230275520097 ) ) ;
#57042=EDGE_LOOP ( 'NONE', ( #68267, #82211, #83672, #28972 ) ) ;
#57043=ORIENTED_EDGE ( 'NONE', *, *, #61264, .F. ) ;
#57044=AXIS2_PLACEMENT_3D ( 'NONE', #7699, #15585, #47007 ) ;
#57045=VECTOR ( 'NONE', #109059, 1000.000000000000000 ) ;
#57046=DIRECTION ( 'NONE',  ( 0.000000000000000000, 1.000000000000000000, 0.000000000000000000 ) ) ;
#57047=LINE ( 'NONE', #5377, #96055 ) ;
#57048=CARTESIAN_POINT ( 'NONE',  ( 0.6499999999999566125, 12.50000000000000000, -6.148780366869526226 ) ) ;
#57049=CIRCLE ( 'NONE', #115527, 0.06509327318403745899 ) ;
#57050=DIRECTION ( 'NONE',  ( -0.000000000000000000, -1.000000000000000000, -0.000000000000000000 ) ) ;
#57051=VECTOR ( 'NONE', #18897, 1000.000000000000000 ) ;
#57052=AXIS2_PLACEMENT_3D ( 'NONE', #75219, #105331, #35942 ) ;
#57053=CARTESIAN_POINT ( 'NONE',  ( 4.799999999999935874, 2.500000000000000000, 0.4464101615137735513 ) ) ;
#57054=VERTEX_POINT ( 'NONE', #23232 ) ;
#57055=CONICAL_SURFACE ( 'NONE', #59236, 0.09999999999999982514, 0.003490658503988666988 ) ;
#57056=DIRECTION ( 'NONE',  ( 0.000000000000000000, -0.9999939076577903929, 0.003490651415223739937 ) ) ;
#57057=ORIENTED_EDGE ( 'NONE', *, *, #123892, .T. ) ;
#57058=CARTESIAN_POINT ( 'NONE',  ( 0.4499999999999569344, 12.50000000000000000, -2.165063509461101710 ) ) ;
#57059=EDGE_CURVE ( 'NONE', #180, #95907, #63163, .T. ) ;
#57060=ORIENTED_EDGE ( 'NONE', *, *, #87244, .F. ) ;
#57061=CIRCLE ( 'NONE', #50818, 0.06509327318403745899 ) ;
#57063=ORIENTED_EDGE ( 'NONE', *, *, #54461, .T. ) ;
#57064=ADVANCED_FACE ( 'NONE', ( #105675 ), #90292, .T. ) ;
#57065=ORIENTED_EDGE ( 'NONE', *, *, #104277, .F. ) ;
#57066=EDGE_CURVE ( 'NONE', #102156, #114764, #13409, .T. ) ;
#57067=DIRECTION ( 'NONE',  ( 0.000000000000000000, 1.000000000000000000, 0.000000000000000000 ) ) ;
#57068=DIRECTION ( 'NONE',  ( 0.000000000000000000, 0.000000000000000000, 1.000000000000000000 ) ) ;
#57069=CARTESIAN_POINT ( 'NONE',  ( -1.850000000000033840, 2.500000000000000000, 1.918653347947321564 ) ) ;
#57070=FACE_OUTER_BOUND ( 'NONE', #25360, .T. ) ;
#57071=EDGE_CURVE ( 'NONE', #22838, #7097, #35647, .T. ) ;
#57072=DIRECTION ( 'NONE',  ( -0.000000000000000000, -1.000000000000000000, -0.000000000000000000 ) ) ;
#57073=ADVANCED_FACE ( 'NONE', ( #73618 ), #43547, .T. ) ;
#57074=ORIENTED_EDGE ( 'NONE', *, *, #74654, .T. ) ;
#57075=DIRECTION ( 'NONE',  ( 0.000000000000000000, -0.9999939076577903929, 0.003490651415223739937 ) ) ;
#57076=DIRECTION ( 'NONE',  ( 0.000000000000000000, 1.000000000000000000, 0.000000000000000000 ) ) ;
#57077=VECTOR ( 'NONE', #12446, 1000.000000000000000 ) ;
#57078=EDGE_CURVE ( 'NONE', #14684, #67886, #42207, .T. ) ;
#57079=CARTESIAN_POINT ( 'NONE',  ( 5.399999999999933742, 2.500000000000000000, -2.385244779468109755E-15 ) ) ;
#57080=EDGE_CURVE ( 'NONE', #39251, #25440, #121605, .T. ) ;
#57082=CARTESIAN_POINT ( 'NONE',  ( -13.34999999999999076, 12.50000000000000000, 2.922977105672690534 ) ) ;
#57083=CARTESIAN_POINT ( 'NONE',  ( 8.349999999999923261, 2.500000000000000000, 1.472243186433545459 ) ) ;
#57084=VERTEX_POINT ( 'NONE', #112913 ) ;
#57085=CIRCLE ( 'NONE', #36179, 0.06509327318403745899 ) ;
#57086=AXIS2_PLACEMENT_3D ( 'NONE', #104321, #53303, #71640 ) ;
#57087=ORIENTED_EDGE ( 'NONE', *, *, #20197, .T. ) ;
#57088=CIRCLE ( 'NONE', #21588, 0.06509327318403745899 ) ;
#57089=CONICAL_SURFACE ( 'NONE', #36183, 0.1000000000000002554, 0.003490658503988666988 ) ;
#57090=FACE_OUTER_BOUND ( 'NONE', #73267, .T. ) ;
#57091=EDGE_CURVE ( 'NONE', #123590, #20895, #50598, .T. ) ;
#57092=ORIENTED_EDGE ( 'NONE', *, *, #20632, .T. ) ;
#57093=DIRECTION ( 'NONE',  ( 0.000000000000000000, -0.000000000000000000, 1.000000000000000000 ) ) ;
#57094=DIRECTION ( 'NONE',  ( 0.000000000000000000, 0.000000000000000000, 1.000000000000000000 ) ) ;
#57095=ADVANCED_FACE ( 'NONE', ( #95855 ), #123741, .T. ) ;
#57096=AXIS2_PLACEMENT_3D ( 'NONE', #20722, #90082, #119546 ) ;
#57097=AXIS2_PLACEMENT_3D ( 'NONE', #31717, #91923, #112212 ) ;
#57098=AXIS2_PLACEMENT_3D ( 'NONE', #33236, #31932, #53508 ) ;
#57099=AXIS2_PLACEMENT_3D ( 'NONE', #68166, #126462, #36799 ) ;
#57100=ORIENTED_EDGE ( 'NONE', *, *, #26242, .F. ) ;
#57102=CARTESIAN_POINT ( 'NONE',  ( -3.950000000000029932, 12.50000000000000000, -6.148780366869526226 ) ) ;
#57103=CARTESIAN_POINT ( 'NONE',  ( -0.4000000000000401013, 12.50000000000000000, -3.702399969078687292 ) ) ;
#57104=CARTESIAN_POINT ( 'NONE',  ( 2.099999999999950351, 2.500000000000000000, -0.6928203230275541413 ) ) ;
#57105=CARTESIAN_POINT ( 'NONE',  ( -7.900000000000011013, 2.500000000000000000, 3.737306695894644371 ) ) ;
#57106=ORIENTED_EDGE ( 'NONE', *, *, #811, .F. ) ;
#57107=CIRCLE ( 'NONE', #101027, 0.06509327318403741736 ) ;
#57108=CARTESIAN_POINT ( 'NONE',  ( 4.999999999999938716, 12.50000000000000000, -5.022947341949754119 ) ) ;
#57110=ORIENTED_EDGE ( 'NONE', *, *, #74520, .F. ) ;
#57112=DIRECTION ( 'NONE',  ( 0.000000000000000000, -0.000000000000000000, 1.000000000000000000 ) ) ;
#57113=PLANE ( 'NONE',  #124319 ) ;
#57114=AXIS2_PLACEMENT_3D ( 'NONE', #122648, #52610, #42832 ) ;
#57115=ORIENTED_EDGE ( 'NONE', *, *, #117922, .T. ) ;
#57116=CARTESIAN_POINT ( 'NONE',  ( 6.849999999999929479, 12.50000000000000000, 6.841600689897072485 ) ) ;
#57117=ORIENTED_EDGE ( 'NONE', *, *, #43195, .T. ) ;
#57118=ADVANCED_FACE ( 'NONE', ( #55285 ), #115325, .T. ) ;
#57119=LINE ( 'NONE', #108150, #48027 ) ;
#57120=CARTESIAN_POINT ( 'NONE',  ( -7.700000000000014388, 2.500000000000000000, -0.3464101615137782364 ) ) ;
#57121=CARTESIAN_POINT ( 'NONE',  ( 9.799999999999913669, 12.50000000000000000, -4.048810130592463530 ) ) ;
#57122=CIRCLE ( 'NONE', #100834, 2.000000000000000000 ) ;
#57123=ADVANCED_FACE ( 'NONE', ( #44830 ), #2467, .T. ) ;
#57124=ORIENTED_EDGE ( 'NONE', *, *, #10403, .F. ) ;
#57125=CARTESIAN_POINT ( 'NONE',  ( -10.85000000000000142, 2.500000000000000000, 2.165063509461097713 ) ) ;
#57126=ADVANCED_FACE ( 'NONE', ( #65078 ), #5516, .T. ) ;
#57128=VERTEX_POINT ( 'NONE', #83471 ) ;
#57129=DIRECTION ( 'NONE',  ( 0.000000000000000000, 1.000000000000000000, 0.000000000000000000 ) ) ;
#57130=EDGE_CURVE ( 'NONE', #63832, #83854, #69375, .T. ) ;
#57131=AXIS2_PLACEMENT_3D ( 'NONE', #90948, #59586, #20918 ) ;
#57132=ORIENTED_EDGE ( 'NONE', *, *, #24549, .F. ) ;
#57133=AXIS2_PLACEMENT_3D ( 'NONE', #122278, #60772, #61433 ) ;
#57134=CARTESIAN_POINT ( 'NONE',  ( 3.149999999999946176, 12.50000000000000000, -6.776507416713039689 ) ) ;
#57135=EDGE_CURVE ( 'NONE', #35861, #129348, #54690, .T. ) ;
#57136=AXIS2_PLACEMENT_3D ( 'NONE', #27890, #48179, #18711 ) ;
#57137=AXIS2_PLACEMENT_3D ( 'NONE', #122477, #23618, #111331 ) ;
#57138=EDGE_CURVE ( 'NONE', #96874, #21203, #67667, .T. ) ;
#57139=ORIENTED_EDGE ( 'NONE', *, *, #78096, .T. ) ;
#57140=DIRECTION ( 'NONE',  ( 0.000000000000000000, 0.000000000000000000, 1.000000000000000000 ) ) ;
#57141=CARTESIAN_POINT ( 'NONE',  ( 8.349999999999919709, 2.500000000000000000, -2.957883832488653830 ) ) ;
#57142=EDGE_LOOP ( 'NONE', ( #82712, #27211, #21899, #79030 ) ) ;
#57143=ORIENTED_EDGE ( 'NONE', *, *, #102644, .F. ) ;
#57144=AXIS2_PLACEMENT_3D ( 'NONE', #49788, #113035, #74407 ) ;
#57145=CARTESIAN_POINT ( 'NONE',  ( 2.699999999999947331, 12.50000000000000000, -4.676537180435978769 ) ) ;
#57146=DIRECTION ( 'NONE',  ( 0.000000000000000000, 0.000000000000000000, 1.000000000000000000 ) ) ;
#57147=VERTEX_POINT ( 'NONE', #27113 ) ;
#57148=EDGE_CURVE ( 'NONE', #126044, #46262, #116125, .T. ) ;
#57149=DIRECTION ( 'NONE',  ( 0.000000000000000000, 0.000000000000000000, -1.000000000000000000 ) ) ;
#57150=DIRECTION ( 'NONE',  ( 0.000000000000000000, 0.000000000000000000, -1.000000000000000000 ) ) ;
#57151=AXIS2_PLACEMENT_3D ( 'NONE', #128662, #10753, #31095 ) ;
#57152=AXIS2_PLACEMENT_3D ( 'NONE', #86688, #126630, #14703 ) ;
#57153=DIRECTION ( 'NONE',  ( 0.000000000000000000, 0.000000000000000000, 1.000000000000000000 ) ) ;
#57154=CARTESIAN_POINT ( 'NONE',  ( -11.64999999999999680, 2.500000000000000000, 2.857883832488649301 ) ) ;
#57156=CARTESIAN_POINT ( 'NONE',  ( -1.650000000000034328, 2.500000000000000000, -6.395190528383301931 ) ) ;
#57157=ORIENTED_EDGE ( 'NONE', *, *, #75378, .F. ) ;
#57158=ORIENTED_EDGE ( 'NONE', *, *, #25963, .F. ) ;
#57160=ORIENTED_EDGE ( 'NONE', *, *, #11190, .T. ) ;
#57161=CARTESIAN_POINT ( 'NONE',  ( -4.400000000000025224, 2.500000000000000000, 4.676537180435972552 ) ) ;
#57162=DIRECTION ( 'NONE',  ( 0.000000000000000000, 0.000000000000000000, -1.000000000000000000 ) ) ;
#57163=DIRECTION ( 'NONE',  ( 0.000000000000000000, 0.000000000000000000, -1.000000000000000000 ) ) ;
#57164=ORIENTED_EDGE ( 'NONE', *, *, #102136, .F. ) ;
#57165=FACE_BOUND ( 'NONE', #100321, .T. ) ;
#57166=EDGE_CURVE ( 'NONE', #125289, #118069, #63124, .T. ) ;
#57167=CARTESIAN_POINT ( 'NONE',  ( 2.299999999999949640, 12.50000000000000000, -0.2813168883297408329 ) ) ;
#57168=DIRECTION ( 'NONE',  ( 0.000000000000000000, 0.000000000000000000, 1.000000000000000000 ) ) ;
#57169=CARTESIAN_POINT ( 'NONE',  ( 1.849999999999950573, 12.50000000000000000, 2.576566944158910744 ) ) ;
#57170=CARTESIAN_POINT ( 'NONE',  ( 11.04999999999991189, 2.500000000000000000, -2.411473670974877859 ) ) ;
#57172=FACE_OUTER_BOUND ( 'NONE', #104861, .T. ) ;
#57173=FACE_OUTER_BOUND ( 'NONE', #95159, .T. ) ;
#57174=CARTESIAN_POINT ( 'NONE',  ( -13.94999999999998685, 2.500000000000000000, 1.818653347947325472 ) ) ;
#57175=CIRCLE ( 'NONE', #38313, 0.06509327318403745899 ) ;
#57176=CONICAL_SURFACE ( 'NONE', #90617, 0.1000000000000002554, 0.003490658503988666988 ) ;
#57177=DIRECTION ( 'NONE',  ( -0.000000000000000000, 1.000000000000000000, -0.000000000000000000 ) ) ;
#57178=DIRECTION ( 'NONE',  ( 0.000000000000000000, -0.9999939076577903929, 0.003490651415223739937 ) ) ;
#57179=CIRCLE ( 'NONE', #59262, 0.1000000000000002554 ) ;
#57180=CIRCLE ( 'NONE', #73905, 0.09999999999999982514 ) ;
#57181=ORIENTED_EDGE ( 'NONE', *, *, #551, .T. ) ;
#57182=ORIENTED_EDGE ( 'NONE', *, *, #47335, .F. ) ;
#57183=EDGE_CURVE ( 'NONE', #125596, #68600, #46384, .T. ) ;
#57184=ORIENTED_EDGE ( 'NONE', *, *, #62911, .T. ) ;
#57185=CIRCLE ( 'NONE', #124077, 0.09999999999999982514 ) ;
#57187=CARTESIAN_POINT ( 'NONE',  ( 17.50000000000010658, -2.362777783881773175, -3.757134105505308685 ) ) ;
#57188=CIRCLE ( 'NONE', #73907, 0.1000000000000002554 ) ;
#57189=AXIS2_PLACEMENT_3D ( 'NONE', #117413, #38256, #89279 ) ;
#57190=CARTESIAN_POINT ( 'NONE',  ( -2.100000000000034728, 2.500000000000000000, 4.330127018922196314 ) ) ;
#57191=EDGE_LOOP ( 'NONE', ( #35283, #81760 ) ) ;
#57192=ORIENTED_EDGE ( 'NONE', *, *, #62469, .T. ) ;
#57193=ORIENTED_EDGE ( 'NONE', *, *, #124165, .F. ) ;
#57194=DIRECTION ( 'NONE',  ( -0.000000000000000000, 1.000000000000000000, -0.000000000000000000 ) ) ;
#57195=AXIS2_PLACEMENT_3D ( 'NONE', #55003, #126335, #53717 ) ;
#57196=VECTOR ( 'NONE', #78793, 1000.000000000000000 ) ;
#57197=AXIS2_PLACEMENT_3D ( 'NONE', #122668, #33023, #23170 ) ;
#57198=CARTESIAN_POINT ( 'NONE',  ( 8.549999999999918998, 2.500000000000000000, -1.818653347947326138 ) ) ;
#57199=FACE_OUTER_BOUND ( 'NONE', #848, .T. ) ;
#57202=AXIS2_PLACEMENT_3D ( 'NONE', #84442, #34056, #113911 ) ;
#57203=EDGE_CURVE ( 'NONE', #45959, #90163, #87940, .T. ) ;
#57204=ORIENTED_EDGE ( 'NONE', *, *, #115021, .F. ) ;
#57205=DIRECTION ( 'NONE',  ( 0.000000000000000000, 0.000000000000000000, 1.000000000000000000 ) ) ;
#57206=EDGE_LOOP ( 'NONE', ( #3580, #124623, #1484, #85299 ) ) ;
#57207=EDGE_LOOP ( 'NONE', ( #90059, #24343, #118054, #3441 ) ) ;
#57208=ORIENTED_EDGE ( 'NONE', *, *, #24356, .F. ) ;
#57209=DIRECTION ( 'NONE',  ( 0.000000000000000000, 1.000000000000000000, 0.000000000000000000 ) ) ;
#57210=ORIENTED_EDGE ( 'NONE', *, *, #125522, .F. ) ;
#57212=CIRCLE ( 'NONE', #111593, 0.09999999999999982514 ) ;
#57213=CARTESIAN_POINT ( 'NONE',  ( -4.800000000000024691, 12.50000000000000000, 4.741630453620009789 ) ) ;
#57214=DIRECTION ( 'NONE',  ( -0.000000000000000000, 1.000000000000000000, -0.000000000000000000 ) ) ;
#57215=DIRECTION ( 'NONE',  ( -0.000000000000000000, 1.000000000000000000, -0.000000000000000000 ) ) ;
#57216=CARTESIAN_POINT ( 'NONE',  ( -3.350000000000028955, 2.500000000000000000, -2.065063509461102065 ) ) ;
#57217=DIRECTION ( 'NONE',  ( -0.000000000000000000, -1.000000000000000000, -0.000000000000000000 ) ) ;
#57218=VECTOR ( 'NONE', #17329, 1000.000000000000000 ) ;
#57219=VERTEX_POINT ( 'NONE', #127888 ) ;
#57220=LINE ( 'NONE', #7465, #51217 ) ;
#57221=AXIS2_PLACEMENT_3D ( 'NONE', #92404, #20460, #42701 ) ;
#57222=CIRCLE ( 'NONE', #44717, 0.06509327318403745899 ) ;
#57223=ORIENTED_EDGE ( 'NONE', *, *, #10316, .T. ) ;
#57224=ADVANCED_FACE ( 'NONE', ( #37590 ), #10954, .T. ) ;
#57225=ORIENTED_EDGE ( 'NONE', *, *, #54864, .T. ) ;
#57226=CARTESIAN_POINT ( 'NONE',  ( -6.071532165918824830E-15, 12.50000000000000000, -4.265033745738164406 ) ) ;
#57227=FACE_OUTER_BOUND ( 'NONE', #4863, .T. ) ;
#57228=ORIENTED_EDGE ( 'NONE', *, *, #8312, .T. ) ;
#57230=DIRECTION ( 'NONE',  ( 0.000000000000000000, 0.000000000000000000, 1.000000000000000000 ) ) ;
#57231=CIRCLE ( 'NONE', #30055, 0.06509327318403745899 ) ;
#57232=ORIENTED_EDGE ( 'NONE', *, *, #30386, .T. ) ;
#57233=AXIS2_PLACEMENT_3D ( 'NONE', #29866, #69785, #77662 ) ;
#57234=AXIS2_PLACEMENT_3D ( 'NONE', #36928, #8090, #48677 ) ;
#57235=EDGE_CURVE ( 'NONE', #59940, #80507, #100855, .T. ) ;
#57236=AXIS2_PLACEMENT_3D ( 'NONE', #99938, #11541, #60664 ) ;
#57237=CARTESIAN_POINT ( 'NONE',  ( -6.900000000000015454, 2.500000000000000000, 4.676537180435972552 ) ) ;
#57238=ORIENTED_EDGE ( 'NONE', *, *, #52833, .T. ) ;
#57239=EDGE_CURVE ( 'NONE', #98343, #71326, #69464, .T. ) ;
#57240=EDGE_CURVE ( 'NONE', #47265, #55655, #92457, .T. ) ;
#57241=VERTEX_POINT ( 'NONE', #108244 ) ;
#57242=CARTESIAN_POINT ( 'NONE',  ( -9.400000000000007461, 12.50000000000000000, 0.4115034346978109769 ) ) ;
#57243=DIRECTION ( 'NONE',  ( 0.000000000000000000, 0.000000000000000000, 1.000000000000000000 ) ) ;
#57244=ADVANCED_FACE ( 'NONE', ( #46760 ), #44434, .T. ) ;
#57246=CONICAL_SURFACE ( 'NONE', #119937, 0.1000000000000002554, 0.003490658503988666988 ) ;
#57247=EDGE_CURVE ( 'NONE', #11699, #104109, #59163, .T. ) ;
#57248=DIRECTION ( 'NONE',  ( -4.274815082592931898E-19, -0.9999939076577903929, -0.003490651415223739937 ) ) ;
#57249=DIRECTION ( 'NONE',  ( 0.000000000000000000, 1.000000000000000000, 0.000000000000000000 ) ) ;
#57250=AXIS2_PLACEMENT_3D ( 'NONE', #59071, #89170, #59736 ) ;
#57251=ADVANCED_FACE ( 'NONE', ( #6788 ), #61161, .T. ) ;
#57252=CONICAL_SURFACE ( 'NONE', #103217, 0.1000000000000002554, 0.003490658503988666988 ) ;
#57253=AXIS2_PLACEMENT_3D ( 'NONE', #97284, #18071, #39046 ) ;
#57254=CARTESIAN_POINT ( 'NONE',  ( 0.1999999999999636513, 2.500000000000000000, -0.4464101615137760493 ) ) ;
#57255=EDGE_CURVE ( 'NONE', #126313, #92073, #113385, .T. ) ;
#57256=EDGE_CURVE ( 'NONE', #112457, #52060, #71617, .T. ) ;
#57257=EDGE_LOOP ( 'NONE', ( #27046, #518 ) ) ;
#57258=CIRCLE ( 'NONE', #53059, 0.06509327318403745899 ) ;
#57259=EDGE_CURVE ( 'NONE', #105130, #27833, #104960, .T. ) ;
#57260=LINE ( 'NONE', #55956, #52747 ) ;
#57261=PLANE ( 'NONE',  #47933 ) ;
#57262=ADVANCED_FACE ( 'NONE', ( #125939 ), #26472, .T. ) ;
#57263=ORIENTED_EDGE ( 'NONE', *, *, #72734, .F. ) ;
#57264=FACE_OUTER_BOUND ( 'NONE', #91831, .T. ) ;
#57265=CARTESIAN_POINT ( 'NONE',  ( -7.950000000000009059, 2.500000000000000000, 6.395190528383296602 ) ) ;
#57266=FACE_OUTER_BOUND ( 'NONE', #72575, .T. ) ;
#57267=FACE_OUTER_BOUND ( 'NONE', #129309, .T. ) ;
#57268=EDGE_CURVE ( 'NONE', #91341, #96622, #16624, .T. ) ;
#57269=LINE ( 'NONE', #62749, #76698 ) ;
#57270=VERTEX_POINT ( 'NONE', #116769 ) ;
#57271=CARTESIAN_POINT ( 'NONE',  ( 11.64999999999990443, 2.500000000000000000, -7.188010851410854052 ) ) ;
#57272=CARTESIAN_POINT ( 'NONE',  ( -13.54999999999998828, 12.50000000000000000, -2.446380397790838046 ) ) ;
#57273=VECTOR ( 'NONE', #24174, 1000.000000000000000 ) ;
#57274=VERTEX_POINT ( 'NONE', #106942 ) ;
#57275=DIRECTION ( 'NONE',  ( 0.000000000000000000, 0.000000000000000000, 1.000000000000000000 ) ) ;
#57276=CONICAL_SURFACE ( 'NONE', #122137, 0.1000000000000002554, 0.003490658503988666988 ) ;
#57277=VERTEX_POINT ( 'NONE', #57213 ) ;
#57278=CONICAL_SURFACE ( 'NONE', #117906, 0.09999999999999982514, 0.003490658503988666988 ) ;
#57279=ORIENTED_EDGE ( 'NONE', *, *, #40319, .T. ) ;
#57281=DIRECTION ( 'NONE',  ( 0.000000000000000000, 0.000000000000000000, -1.000000000000000000 ) ) ;
#57282=AXIS2_PLACEMENT_3D ( 'NONE', #71053, #43542, #22616 ) ;
#57283=VERTEX_POINT ( 'NONE', #89253 ) ;
#57284=DIRECTION ( 'NONE',  ( 0.000000000000000000, 0.000000000000000000, 1.000000000000000000 ) ) ;
#57285=CARTESIAN_POINT ( 'NONE',  ( -5.850000000000019185, 12.50000000000000000, 2.099970236277060032 ) ) ;
#57286=DIRECTION ( 'NONE',  ( -0.000000000000000000, 1.000000000000000000, -0.000000000000000000 ) ) ;
#57287=AXIS2_PLACEMENT_3D ( 'NONE', #22196, #51011, #1245 ) ;
#57288=ORIENTED_EDGE ( 'NONE', *, *, #10980, .T. ) ;
#57289=VECTOR ( 'NONE', #115963, 1000.000000000000000 ) ;
#57290=AXIS2_PLACEMENT_3D ( 'NONE', #104163, #24956, #84521 ) ;
#57291=FACE_BOUND ( 'NONE', #32962, .T. ) ;
#57292=DIRECTION ( 'NONE',  ( 0.000000000000000000, 0.000000000000000000, 1.000000000000000000 ) ) ;
#57293=VERTEX_POINT ( 'NONE', #101661 ) ;
#57294=VECTOR ( 'NONE', #87646, 1000.000000000000000 ) ;
#57296=DIRECTION ( 'NONE',  ( 0.000000000000000000, 1.000000000000000000, 0.000000000000000000 ) ) ;
#57297=EDGE_LOOP ( 'NONE', ( #47398, #24611 ) ) ;
#57298=EDGE_CURVE ( 'NONE', #112590, #79702, #38180, .T. ) ;
#57299=VERTEX_POINT ( 'NONE', #82006 ) ;
#57300=EDGE_CURVE ( 'NONE', #113115, #86732, #8815, .T. ) ;
#57301=ORIENTED_EDGE ( 'NONE', *, *, #96216, .T. ) ;
#57302=CARTESIAN_POINT ( 'NONE',  ( 4.399999999999939071, 2.500000000000000000, 0.4464101615137736623 ) ) ;
#57303=AXIS2_PLACEMENT_3D ( 'NONE', #68954, #117376, #67656 ) ;
#57304=DIRECTION ( 'NONE',  ( 0.000000000000000000, 1.000000000000000000, 0.000000000000000000 ) ) ;
#57305=DIRECTION ( 'NONE',  ( 0.000000000000000000, 0.000000000000000000, 1.000000000000000000 ) ) ;
#57306=FACE_BOUND ( 'NONE', #93087, .T. ) ;
#57307=ORIENTED_EDGE ( 'NONE', *, *, #55536, .T. ) ;
#57308=CARTESIAN_POINT ( 'NONE',  ( -3.100000000000028511, 12.50000000000000000, -0.2813168883297408329 ) ) ;
#57309=DIRECTION ( 'NONE',  ( 0.000000000000000000, 0.000000000000000000, 1.000000000000000000 ) ) ;
#57310=CONICAL_SURFACE ( 'NONE', #115790, 0.1000000000000002554, 0.003490658503988666988 ) ;
#57311=ORIENTED_EDGE ( 'NONE', *, *, #3181, .F. ) ;
#57312=ADVANCED_FACE ( 'NONE', ( #39545 ), #42294, .T. ) ;
#57313=PLANE ( 'NONE',  #126488 ) ;
#57314=CARTESIAN_POINT ( 'NONE',  ( 2.899999999999944844, 2.500000000000000000, 4.922947341949748257 ) ) ;
#57315=CARTESIAN_POINT ( 'NONE',  ( 9.549999999999918998, 2.500000000000000000, -6.495190528383302464 ) ) ;
#57316=CARTESIAN_POINT ( 'NONE',  ( 8.949999999999919353, 2.500000000000000000, 2.511473670974873507 ) ) ;
#57317=DIRECTION ( 'NONE',  ( -0.000000000000000000, -1.000000000000000000, -0.000000000000000000 ) ) ;
#57318=AXIS2_PLACEMENT_3D ( 'NONE', #50895, #118982, #47189 ) ;
#57319=VECTOR ( 'NONE', #6539, 1000.000000000000000 ) ;
#57320=ORIENTED_EDGE ( 'NONE', *, *, #36725, .T. ) ;
#57321=ORIENTED_EDGE ( 'NONE', *, *, #56900, .F. ) ;
#57322=ORIENTED_EDGE ( 'NONE', *, *, #89431, .T. ) ;
#57323=EDGE_LOOP ( 'NONE', ( #70707, #39486, #123254, #19577 ) ) ;
#57324=ORIENTED_EDGE ( 'NONE', *, *, #74667, .T. ) ;
#57325=LINE ( 'NONE', #7561, #38062 ) ;
#57326=DIRECTION ( 'NONE',  ( 0.000000000000000000, 1.000000000000000000, 0.000000000000000000 ) ) ;
#57327=ORIENTED_EDGE ( 'NONE', *, *, #2846, .T. ) ;
#57328=FACE_BOUND ( 'NONE', #25307, .T. ) ;
#57329=DIRECTION ( 'NONE',  ( -0.000000000000000000, 1.000000000000000000, -0.000000000000000000 ) ) ;
#57330=AXIS2_PLACEMENT_3D ( 'NONE', #90591, #33619, #83985 ) ;
#57331=CARTESIAN_POINT ( 'NONE',  ( -0.8000000000000315747, 2.500000000000000000, 0.000000000000000000 ) ) ;
#57332=DIRECTION ( 'NONE',  ( 0.000000000000000000, 0.000000000000000000, -1.000000000000000000 ) ) ;
#57333=FACE_OUTER_BOUND ( 'NONE', #64727, .T. ) ;
#57334=CARTESIAN_POINT ( 'NONE',  ( -8.350000000000013856, 12.50000000000000000, -7.188010851410848723 ) ) ;
#57335=EDGE_LOOP ( 'NONE', ( #123642, #85581 ) ) ;
#57336=DIRECTION ( 'NONE',  ( 0.000000000000000000, 0.000000000000000000, 1.000000000000000000 ) ) ;
#57337=ORIENTED_EDGE ( 'NONE', *, *, #22342, .T. ) ;
#57338=CIRCLE ( 'NONE', #99117, 0.06509327318403745899 ) ;
#57339=VECTOR ( 'NONE', #10805, 1000.000000000000000 ) ;
#57340=EDGE_LOOP ( 'NONE', ( #74193, #85607, #127744, #108154 ) ) ;
#57341=ORIENTED_EDGE ( 'NONE', *, *, #126225, .T. ) ;
#57342=DIRECTION ( 'NONE',  ( -4.274815082592931898E-19, -0.9999939076577903929, -0.003490651415223739937 ) ) ;
#57344=DIRECTION ( 'NONE',  ( -0.000000000000000000, 1.000000000000000000, -0.000000000000000000 ) ) ;
#57345=ORIENTED_EDGE ( 'NONE', *, *, #5051, .F. ) ;
#57346=CARTESIAN_POINT ( 'NONE',  ( 14.69205215096538097, 2.499999999999999556, -6.336420066640663151 ) ) ;
#57347=AXIS2_PLACEMENT_3D ( 'NONE', #110422, #72442, #51516 ) ;
#57348=DIRECTION ( 'NONE',  ( -0.000000000000000000, -1.000000000000000000, -0.000000000000000000 ) ) ;
#57349=DIRECTION ( 'NONE',  ( 0.000000000000000000, 1.000000000000000000, 0.000000000000000000 ) ) ;
#57351=FACE_OUTER_BOUND ( 'NONE', #116668, .T. ) ;
#57352=LINE ( 'NONE', #118206, #119838 ) ;
#57353=EDGE_CURVE ( 'NONE', #113894, #79929, #2154, .T. ) ;
#57354=LINE ( 'NONE', #75689, #11916 ) ;
#57355=EDGE_CURVE ( 'NONE', #123793, #17546, #110190, .T. ) ;
#57356=ORIENTED_EDGE ( 'NONE', *, *, #127579, .F. ) ;
#57357=CARTESIAN_POINT ( 'NONE',  ( -12.94999999999999218, 2.500000000000000000, -2.065063509461099844 ) ) ;
#57358=ORIENTED_EDGE ( 'NONE', *, *, #55916, .F. ) ;
#57359=AXIS2_PLACEMENT_3D ( 'NONE', #106172, #116621, #66874 ) ;
#57360=ORIENTED_EDGE ( 'NONE', *, *, #48303, .T. ) ;
#57361=DIRECTION ( 'NONE',  ( 0.000000000000000000, 1.000000000000000000, 0.000000000000000000 ) ) ;
#57362=CIRCLE ( 'NONE', #80356, 0.06509327318403745899 ) ;
#57363=VECTOR ( 'NONE', #50158, 1000.000000000000000 ) ;
#57364=LINE ( 'NONE', #19354, #32142 ) ;
#57365=AXIS2_PLACEMENT_3D ( 'NONE', #110462, #20801, #111082 ) ;
#57366=CARTESIAN_POINT ( 'NONE',  ( -4.600000000000028955, 12.50000000000000000, -4.330127018922201643 ) ) ;
#57367=EDGE_CURVE ( 'NONE', #75768, #7162, #94593, .T. ) ;
#57368=ORIENTED_EDGE ( 'NONE', *, *, #100305, .T. ) ;
#57369=ORIENTED_EDGE ( 'NONE', *, *, #32344, .T. ) ;
#57370=DIRECTION ( 'NONE',  ( -0.000000000000000000, 1.000000000000000000, -0.000000000000000000 ) ) ;
#57371=CONICAL_SURFACE ( 'NONE', #51036, 0.09999999999999982514, 0.003490658503988666988 ) ;
#57372=CIRCLE ( 'NONE', #934, 0.1000000000000002554 ) ;
#57373=CIRCLE ( 'NONE', #53184, 0.1000000000000000472 ) ;
#57374=CARTESIAN_POINT ( 'NONE',  ( -12.09999999999999609, 2.500000000000000000, 1.734723475976807094E-15 ) ) ;
#57375=DIRECTION ( 'NONE',  ( 0.000000000000000000, 0.000000000000000000, 1.000000000000000000 ) ) ;
#57376=ORIENTED_EDGE ( 'NONE', *, *, #13824, .F. ) ;
#57377=EDGE_LOOP ( 'NONE', ( #86063, #34550 ) ) ;
#57378=CARTESIAN_POINT ( 'NONE',  ( -1.450000000000035483, 12.50000000000000000, 6.148780366869520897 ) ) ;
#57379=EDGE_LOOP ( 'NONE', ( #106761, #98619, #95180, #41784 ) ) ;
#57380=CARTESIAN_POINT ( 'NONE',  ( 1.699999999999950218, 12.50000000000000000, 4.330127018922196314 ) ) ;
#57381=CIRCLE ( 'NONE', #78328, 0.06509327318403745899 ) ;
#57383=CARTESIAN_POINT ( 'NONE',  ( 4.149999999999938183, 2.500000000000000000, 7.188010851410848723 ) ) ;
#57384=EDGE_LOOP ( 'NONE', ( #116473, #77846 ) ) ;
#57385=DIRECTION ( 'NONE',  ( -0.000000000000000000, 1.000000000000000000, -0.000000000000000000 ) ) ;
#57386=EDGE_CURVE ( 'NONE', #3394, #111598, #54892, .T. ) ;
#57387=CARTESIAN_POINT ( 'NONE',  ( 2.099999999999950351, 2.500000000000000000, 0.09999999999999772959 ) ) ;
#57388=DIRECTION ( 'NONE',  ( -0.000000000000000000, -1.000000000000000000, -0.000000000000000000 ) ) ;
#57389=AXIS2_PLACEMENT_3D ( 'NONE', #36498, #126796, #106503 ) ;
#57390=DIRECTION ( 'NONE',  ( -0.000000000000000000, -1.000000000000000000, -0.000000000000000000 ) ) ;
#57391=EDGE_LOOP ( 'NONE', ( #22489, #52946 ) ) ;
#57392=ADVANCED_FACE ( 'NONE', ( #109546 ), #125895, .T. ) ;
#57393=FACE_OUTER_BOUND ( 'NONE', #77959, .T. ) ;
#57394=CARTESIAN_POINT ( 'NONE',  ( -3.150000000000029221, 2.500000000000000000, 2.611473670974873151 ) ) ;
#57395=ORIENTED_EDGE ( 'NONE', *, *, #52681, .F. ) ;
#57396=VERTEX_POINT ( 'NONE', #30357 ) ;
#57397=EDGE_CURVE ( 'NONE', #15907, #92009, #29763, .T. ) ;
#57398=EDGE_CURVE ( 'NONE', #24838, #7948, #71528, .T. ) ;
#57399=CARTESIAN_POINT ( 'NONE',  ( 4.799999999999937650, 12.50000000000000000, -4.048810130592463530 ) ) ;
#57400=CARTESIAN_POINT ( 'NONE',  ( -4.600000000000025402, 12.50000000000000000, -2.385244779468109755E-15 ) ) ;
#57401=CARTESIAN_POINT ( 'NONE',  ( 12.04999999999990834, 12.50000000000000000, -2.165063509461101710 ) ) ;
#57404=ADVANCED_FACE ( 'NONE', ( #50609 ), #88224, .T. ) ;
#57405=AXIS2_PLACEMENT_3D ( 'NONE', #57816, #27690, #57162 ) ;
#57406=DIRECTION ( 'NONE',  ( 0.000000000000000000, 1.000000000000000000, 0.000000000000000000 ) ) ;
#57407=DIRECTION ( 'NONE',  ( 0.000000000000000000, 0.000000000000000000, 1.000000000000000000 ) ) ;
#57408=DIRECTION ( 'NONE',  ( -0.000000000000000000, -1.000000000000000000, -0.000000000000000000 ) ) ;
#57409=CARTESIAN_POINT ( 'NONE',  ( 9.549999999999918998, 2.500000000000000000, 2.165063509461097713 ) ) ;
#57410=CARTESIAN_POINT ( 'NONE',  ( -5.200000000000022382, 2.500000000000000000, 4.676537180435972552 ) ) ;
#57411=EDGE_CURVE ( 'NONE', #101516, #42047, #121699, .T. ) ;
#57412=EDGE_CURVE ( 'NONE', #123389, #62648, #81994, .T. ) ;
#57413=CARTESIAN_POINT ( 'NONE',  ( -3.350000000000028511, 12.50000000000000000, 2.792790559304612064 ) ) ;
#57414=CIRCLE ( 'NONE', #969, 0.09999999999999982514 ) ;
#57415=VECTOR ( 'NONE', #107202, 1000.000000000000000 ) ;
#57416=ADVANCED_FACE ( 'NONE', ( #53211 ), #21545, .T. ) ;
#57417=EDGE_CURVE ( 'NONE', #8747, #36304, #75818, .T. ) ;
#57418=ORIENTED_EDGE ( 'NONE', *, *, #19203, .F. ) ;
#57419=CARTESIAN_POINT ( 'NONE',  ( 11.64999999999990798, 12.50000000000000000, 7.188010851410848723 ) ) ;
#57420=ADVANCED_FACE ( 'NONE', ( #115301 ), #109272, .T. ) ;
#57421=CARTESIAN_POINT ( 'NONE',  ( 10.84999999999990905, 12.50000000000000000, -5.802370205355749988 ) ) ;
#57422=DIRECTION ( 'NONE',  ( 0.000000000000000000, 1.000000000000000000, 0.000000000000000000 ) ) ;
#57423=CARTESIAN_POINT ( 'NONE',  ( -9.200000000000006395, 2.500000000000000000, 4.330127018922196314 ) ) ;
#57425=ORIENTED_EDGE ( 'NONE', *, *, #91988, .T. ) ;
#57426=CARTESIAN_POINT ( 'NONE',  ( -4.600000000000025402, 2.500000000000000000, 4.330127018922196314 ) ) ;
#57427=AXIS2_PLACEMENT_3D ( 'NONE', #124577, #66921, #8637 ) ;
#57429=CARTESIAN_POINT ( 'NONE',  ( 6.049999999999934097, 12.50000000000000000, 6.213873640053559022 ) ) ;
#57430=CARTESIAN_POINT ( 'NONE',  ( 2.899999999999945732, 12.50000000000000000, -4.265033745738164406 ) ) ;
#57431=ORIENTED_EDGE ( 'NONE', *, *, #70681, .F. ) ;
#57432=ORIENTED_EDGE ( 'NONE', *, *, #127000, .T. ) ;
#57433=AXIS2_PLACEMENT_3D ( 'NONE', #64544, #51044, #41865 ) ;
#57434=CIRCLE ( 'NONE', #21856, 0.06509327318403745899 ) ;
#57435=ORIENTED_EDGE ( 'NONE', *, *, #57256, .F. ) ;
#57436=EDGE_LOOP ( 'NONE', ( #62211, #63799 ) ) ;
#57438=DIRECTION ( 'NONE',  ( 0.000000000000000000, 1.000000000000000000, 0.000000000000000000 ) ) ;
#57439=AXIS2_PLACEMENT_3D ( 'NONE', #73120, #73743, #113692 ) ;
#57440=DIRECTION ( 'NONE',  ( -0.000000000000000000, -1.000000000000000000, -0.000000000000000000 ) ) ;
#57441=FACE_OUTER_BOUND ( 'NONE', #83759, .T. ) ;
#57442=AXIS2_PLACEMENT_3D ( 'NONE', #19961, #59907, #103016 ) ;
#57443=DIRECTION ( 'NONE',  ( 0.000000000000000000, 0.000000000000000000, -1.000000000000000000 ) ) ;
#57444=VERTEX_POINT ( 'NONE', #75400 ) ;
#57445=CARTESIAN_POINT ( 'NONE',  ( 5.799999999999934985, 12.50000000000000000, -4.395220292106239768 ) ) ;
#57446=EDGE_LOOP ( 'NONE', ( #76840, #64291 ) ) ;
#57447=CARTESIAN_POINT ( 'NONE',  ( 48.84100846713599253, -2.320798421931173028, -5.300800859552192712 ) ) ;
#57448=DIRECTION ( 'NONE',  ( -0.000000000000000000, -1.000000000000000000, -0.000000000000000000 ) ) ;
#57449=CARTESIAN_POINT ( 'NONE',  ( 0.1999999999999576006, 2.500000000000000000, -4.576537180435978236 ) ) ;
#57450=DIRECTION ( 'NONE',  ( 0.000000000000000000, 1.000000000000000000, 0.000000000000000000 ) ) ;
#57451=DIRECTION ( 'NONE',  ( -0.000000000000000000, -1.000000000000000000, -0.000000000000000000 ) ) ;
#57452=ORIENTED_EDGE ( 'NONE', *, *, #40132, .F. ) ;
#57453=ADVANCED_FACE ( 'NONE', ( #93133 ), #93768, .T. ) ;
#57454=CONICAL_SURFACE ( 'NONE', #3080, 0.09999999999999982514, 0.003490658503988666988 ) ;
#57455=ORIENTED_EDGE ( 'NONE', *, *, #74826, .T. ) ;
#57456=VERTEX_POINT ( 'NONE', #112770 ) ;
#57457=AXIS2_PLACEMENT_3D ( 'NONE', #75110, #16156, #115011 ) ;
#57458=EDGE_CURVE ( 'NONE', #52047, #114100, #90482, .T. ) ;
#57460=DIRECTION ( 'NONE',  ( -4.274815082592931898E-19, -0.9999939076577903929, -0.003490651415223739937 ) ) ;
#57461=DIRECTION ( 'NONE',  ( 0.000000000000000000, -0.9999939076577903929, 0.003490651415223739937 ) ) ;
#57462=AXIS2_PLACEMENT_3D ( 'NONE', #45494, #15348, #94565 ) ;
#57463=VECTOR ( 'NONE', #75679, 1000.000000000000000 ) ;
#57464=DIRECTION ( 'NONE',  ( 0.000000000000000000, 1.000000000000000000, 0.000000000000000000 ) ) ;
#57465=FACE_BOUND ( 'NONE', #71512, .T. ) ;
#57466=DIRECTION ( 'NONE',  ( -4.274815082592931898E-19, -0.9999939076577903929, -0.003490651415223739937 ) ) ;
#57467=DIRECTION ( 'NONE',  ( 0.000000000000000000, -0.000000000000000000, 1.000000000000000000 ) ) ;
#57468=CARTESIAN_POINT ( 'NONE',  ( 13.74999999999989697, 2.500000000000000000, 2.857883832488649301 ) ) ;
#57469=DIRECTION ( 'NONE',  ( 0.000000000000000000, 1.000000000000000000, 0.000000000000000000 ) ) ;
#57470=CONICAL_SURFACE ( 'NONE', #128596, 0.1000000000000002554, 0.003490658503988666988 ) ;
#57471=AXIS2_PLACEMENT_3D ( 'NONE', #71331, #111245, #101458 ) ;
#57472=AXIS2_PLACEMENT_3D ( 'NONE', #47414, #48058, #69616 ) ;
#57474=CIRCLE ( 'NONE', #118096, 0.06509327318403745899 ) ;
#57475=DIRECTION ( 'NONE',  ( -0.000000000000000000, -1.000000000000000000, -0.000000000000000000 ) ) ;
#57476=FACE_OUTER_BOUND ( 'NONE', #12937, .T. ) ;
#57477=AXIS2_PLACEMENT_3D ( 'NONE', #78987, #27932, #47585 ) ;
#57478=AXIS2_PLACEMENT_3D ( 'NONE', #123969, #42877, #44131 ) ;
#57479=DIRECTION ( 'NONE',  ( -0.000000000000000000, -1.000000000000000000, -0.000000000000000000 ) ) ;
#57480=ORIENTED_EDGE ( 'NONE', *, *, #7505, .F. ) ;
#57481=ORIENTED_EDGE ( 'NONE', *, *, #44276, .T. ) ;
#57482=VERTEX_POINT ( 'NONE', #24382 ) ;
#57483=EDGE_LOOP ( 'NONE', ( #123594, #12009 ) ) ;
#57485=DIRECTION ( 'NONE',  ( 0.000000000000000000, 1.000000000000000000, 0.000000000000000000 ) ) ;
#57486=FACE_BOUND ( 'NONE', #123012, .T. ) ;
#57487=CARTESIAN_POINT ( 'NONE',  ( -6.700000000000019718, 12.50000000000000000, -2.385244779468109755E-15 ) ) ;
#57488=DIRECTION ( 'NONE',  ( 0.000000000000000000, 0.000000000000000000, -1.000000000000000000 ) ) ;
#57489=ORIENTED_EDGE ( 'NONE', *, *, #10574, .T. ) ;
#57490=CARTESIAN_POINT ( 'NONE',  ( -8.550000000000007816, 2.500000000000000000, 6.048780366869520364 ) ) ;
#57491=DIRECTION ( 'NONE',  ( -0.000000000000000000, 1.000000000000000000, -0.000000000000000000 ) ) ;
#57492=DIRECTION ( 'NONE',  ( 0.000000000000000000, 1.000000000000000000, 0.000000000000000000 ) ) ;
#57493=AXIS2_PLACEMENT_3D ( 'NONE', #30946, #108829, #19148 ) ;
#57494=ORIENTED_EDGE ( 'NONE', *, *, #104305, .F. ) ;
#57495=CARTESIAN_POINT ( 'NONE',  ( 10.64999999999990976, 12.50000000000000000, 2.576566944158910744 ) ) ;
#57496=CARTESIAN_POINT ( 'NONE',  ( -12.49999999999999289, 2.500000000000000000, -0.6928203230275500335 ) ) ;
#57497=EDGE_CURVE ( 'NONE', #44808, #93899, #44670, .T. ) ;
#57500=EDGE_LOOP ( 'NONE', ( #36276, #89612, #10431, #101732 ) ) ;
#57501=LINE ( 'NONE', #126236, #27817 ) ;
#57502=DIRECTION ( 'NONE',  ( 0.000000000000000000, -0.000000000000000000, 1.000000000000000000 ) ) ;
#57503=CIRCLE ( 'NONE', #90952, 0.06509327318403745899 ) ;
#57504=CIRCLE ( 'NONE', #28258, 0.09999999999999982514 ) ;
#57505=ORIENTED_EDGE ( 'NONE', *, *, #80339, .T. ) ;
#57506=DIRECTION ( 'NONE',  ( -0.000000000000000000, 1.000000000000000000, -0.000000000000000000 ) ) ;
#57507=CARTESIAN_POINT ( 'NONE',  ( -8.350000000000008527, 12.50000000000000000, 7.188010851410848723 ) ) ;
#57509=DIRECTION ( 'NONE',  ( -4.274815082592931898E-19, -0.9999939076577903929, -0.003490651415223739937 ) ) ;
#57510=ORIENTED_EDGE ( 'NONE', *, *, #127819, .T. ) ;
#57511=EDGE_CURVE ( 'NONE', #46085, #11888, #46575, .T. ) ;
#57512=ORIENTED_EDGE ( 'NONE', *, *, #60044, .T. ) ;
#57513=ADVANCED_FACE ( 'NONE', ( #4709 ), #34867, .T. ) ;
#57514=DIRECTION ( 'NONE',  ( -0.000000000000000000, -1.000000000000000000, -0.000000000000000000 ) ) ;
#57515=ORIENTED_EDGE ( 'NONE', *, *, #106421, .T. ) ;
#57516=FACE_OUTER_BOUND ( 'NONE', #29565, .T. ) ;
#57517=FACE_BOUND ( 'NONE', #126167, .T. ) ;
#57518=AXIS2_PLACEMENT_3D ( 'NONE', #49252, #119252, #51182 ) ;
#57520=AXIS2_PLACEMENT_3D ( 'NONE', #18197, #37843, #49622 ) ;
#57522=VERTEX_POINT ( 'NONE', #33568 ) ;
#57523=LINE ( 'NONE', #16273, #100564 ) ;
#57524=PLANE ( 'NONE',  #90425 ) ;
#57525=FACE_OUTER_BOUND ( 'NONE', #74535, .T. ) ;
#57526=DIRECTION ( 'NONE',  ( -0.000000000000000000, 1.000000000000000000, -0.000000000000000000 ) ) ;
#57527=EDGE_CURVE ( 'NONE', #26026, #81857, #73759, .T. ) ;
#57528=CARTESIAN_POINT ( 'NONE',  ( -3.550000000000028244, 12.50000000000000000, 2.511473670974873507 ) ) ;
#57529=ORIENTED_EDGE ( 'NONE', *, *, #5098, .F. ) ;
#57530=VERTEX_POINT ( 'NONE', #10377 ) ;
#57531=CARTESIAN_POINT ( 'NONE',  ( 4.599999999999938360, 12.50000000000000000, -2.276824562219559311E-15 ) ) ;
#57532=CONICAL_SURFACE ( 'NONE', #84708, 0.1000000000000002554, 0.003490658503988666988 ) ;
#57533=DIRECTION ( 'NONE',  ( 0.000000000000000000, 0.000000000000000000, -1.000000000000000000 ) ) ;
#57534=CARTESIAN_POINT ( 'NONE',  ( 5.199999999999935341, 2.500000000000000000, -3.983716857408426293 ) ) ;
#57535=ORIENTED_EDGE ( 'NONE', *, *, #105946, .T. ) ;
#57536=VERTEX_POINT ( 'NONE', #30684 ) ;
#57537=ORIENTED_EDGE ( 'NONE', *, *, #18951, .F. ) ;
#57538=DIRECTION ( 'NONE',  ( 0.000000000000000000, 1.000000000000000000, 0.000000000000000000 ) ) ;
#57539=DIRECTION ( 'NONE',  ( 0.000000000000000000, 1.000000000000000000, 0.000000000000000000 ) ) ;
#57540=DIRECTION ( 'NONE',  ( 0.000000000000000000, -0.9999939076577903929, 0.003490651415223739937 ) ) ;
#57541=DIRECTION ( 'NONE',  ( 0.000000000000000000, 0.000000000000000000, 1.000000000000000000 ) ) ;
#57542=FACE_OUTER_BOUND ( 'NONE', #98511, .T. ) ;
#57544=DIRECTION ( 'NONE',  ( 0.000000000000000000, 0.000000000000000000, 1.000000000000000000 ) ) ;
#57545=DIRECTION ( 'NONE',  ( -0.000000000000000000, -1.000000000000000000, -0.000000000000000000 ) ) ;
#57546=CONICAL_SURFACE ( 'NONE', #28298, 0.1000000000000002554, 0.003490658503988666988 ) ;
#57547=DIRECTION ( 'NONE',  ( 0.000000000000000000, 1.000000000000000000, 0.000000000000000000 ) ) ;
#57549=ORIENTED_EDGE ( 'NONE', *, *, #82126, .T. ) ;
#57550=EDGE_CURVE ( 'NONE', #45421, #92599, #113474, .T. ) ;
#57551=AXIS2_PLACEMENT_3D ( 'NONE', #59934, #12091, #10170 ) ;
#57553=DIRECTION ( 'NONE',  ( -0.000000000000000000, -1.000000000000000000, -0.000000000000000000 ) ) ;
#57554=CIRCLE ( 'NONE', #3178, 0.06509327318403745899 ) ;
#57555=EDGE_LOOP ( 'NONE', ( #96576, #93504, #42002, #47399 ) ) ;
#57556=ORIENTED_EDGE ( 'NONE', *, *, #44828, .F. ) ;
#57557=EDGE_CURVE ( 'NONE', #42124, #46460, #57033, .T. ) ;
#57558=DIRECTION ( 'NONE',  ( 0.000000000000000000, 0.000000000000000000, 1.000000000000000000 ) ) ;
#57559=CARTESIAN_POINT ( 'NONE',  ( 2.299999999999946976, 2.500000000000000000, 4.676537180435972552 ) ) ;
#57560=DIRECTION ( 'NONE',  ( -4.274815082592931898E-19, -0.9999939076577903929, -0.003490651415223739937 ) ) ;
#57561=EDGE_CURVE ( 'NONE', #18141, #26625, #107217, .T. ) ;
#57562=CONICAL_SURFACE ( 'NONE', #55498, 0.1000000000000002554, 0.003490658503988666988 ) ;
#57563=DIRECTION ( 'NONE',  ( 0.000000000000000000, 0.000000000000000000, 1.000000000000000000 ) ) ;
#57564=CIRCLE ( 'NONE', #124453, 0.06509327318403745899 ) ;
#57566=CARTESIAN_POINT ( 'NONE',  ( 2.899999999999943956, 2.500000000000000000, 4.330127018922196314 ) ) ;
#57567=CARTESIAN_POINT ( 'NONE',  ( -1.450000000000036371, 2.500000000000000000, 2.511473670974873507 ) ) ;
#57568=DIRECTION ( 'NONE',  ( 0.000000000000000000, 0.000000000000000000, -1.000000000000000000 ) ) ;
#57569=ORIENTED_EDGE ( 'NONE', *, *, #109997, .F. ) ;
#57570=DIRECTION ( 'NONE',  ( 0.000000000000000000, 0.000000000000000000, 1.000000000000000000 ) ) ;
#57571=ADVANCED_FACE ( 'NONE', ( #30035 ), #50307, .T. ) ;
#57572=CIRCLE ( 'NONE', #1114, 0.09999999999999999167 ) ;
#57573=EDGE_CURVE ( 'NONE', #97417, #56205, #40509, .T. ) ;
#57574=EDGE_CURVE ( 'NONE', #19384, #99701, #120338, .T. ) ;
#57575=EDGE_CURVE ( 'NONE', #115572, #120080, #118391, .T. ) ;
#57576=CARTESIAN_POINT ( 'NONE',  ( -12.89999999999999147, 12.50000000000000000, 5.088040615133786027 ) ) ;
#57577=AXIS2_PLACEMENT_3D ( 'NONE', #14717, #35676, #124045 ) ;
#57578=CIRCLE ( 'NONE', #84754, 0.06509327318403745899 ) ;
#57579=ORIENTED_EDGE ( 'NONE', *, *, #27853, .T. ) ;
#57580=EDGE_CURVE ( 'NONE', #88147, #102605, #50794, .T. ) ;
#57581=ORIENTED_EDGE ( 'NONE', *, *, #118544, .F. ) ;
#57582=AXIS2_PLACEMENT_3D ( 'NONE', #34247, #104877, #34891 ) ;
#57583=ORIENTED_EDGE ( 'NONE', *, *, #87990, .F. ) ;
#57584=VERTEX_POINT ( 'NONE', #69278 ) ;
#57585=DIRECTION ( 'NONE',  ( 0.000000000000000000, 1.000000000000000000, 0.000000000000000000 ) ) ;
#57586=DIRECTION ( 'NONE',  ( -0.000000000000000000, 1.000000000000000000, -0.000000000000000000 ) ) ;
#57587=EDGE_CURVE ( 'NONE', #17997, #81742, #32029, .T. ) ;
#57588=ORIENTED_EDGE ( 'NONE', *, *, #105380, .F. ) ;
#57589=CARTESIAN_POINT ( 'NONE',  ( -10.60000000000000142, 12.50000000000000000, -0.4115034346978156399 ) ) ;
#57590=CARTESIAN_POINT ( 'NONE',  ( 17.50000000000000000, -2.750000000000000000, -9.999999999999998224 ) ) ;
#57591=DIRECTION ( 'NONE',  ( -0.000000000000000000, -1.000000000000000000, -0.000000000000000000 ) ) ;
#57592=ORIENTED_EDGE ( 'NONE', *, *, #119762, .T. ) ;
#57593=DIRECTION ( 'NONE',  ( 0.000000000000000000, 1.000000000000000000, 0.000000000000000000 ) ) ;
#57594=AXIS2_PLACEMENT_3D ( 'NONE', #101612, #83261, #4654 ) ;
#57595=CARTESIAN_POINT ( 'NONE',  ( -13.74999999999995381, 2.500000000000000000, -2.265063509461099578 ) ) ;
#57596=EDGE_LOOP ( 'NONE', ( #39827, #6277 ) ) ;
#57597=VERTEX_POINT ( 'NONE', #109207 ) ;
#57598=EDGE_LOOP ( 'NONE', ( #44855, #1990 ) ) ;
#57599=DIRECTION ( 'NONE',  ( 0.000000000000000000, 1.000000000000000000, 0.000000000000000000 ) ) ;
#57600=CONICAL_SURFACE ( 'NONE', #9470, 0.09999999999999982514, 0.003490658503988666988 ) ;
#57601=AXIS2_PLACEMENT_3D ( 'NONE', #78116, #117349, #38189 ) ;
#57602=DIRECTION ( 'NONE',  ( 0.000000000000000000, -0.000000000000000000, 1.000000000000000000 ) ) ;
#57603=CONICAL_SURFACE ( 'NONE', #99368, 0.09999999999999982514, 0.003490658503988666988 ) ;
#57604=EDGE_LOOP ( 'NONE', ( #65261, #82338, #99304, #22774 ) ) ;
#57606=CARTESIAN_POINT ( 'NONE',  ( -15.79999999999998117, 2.500000000000000000, -0.1000000000000000056 ) ) ;
#57607=CARTESIAN_POINT ( 'NONE',  ( 105.5000000000000142, 0.000000000000000000, 2.000000000000000000 ) ) ;
#57608=DIRECTION ( 'NONE',  ( 0.000000000000000000, 1.000000000000000000, 0.000000000000000000 ) ) ;
#57609=AXIS2_PLACEMENT_3D ( 'NONE', #39297, #107992, #118454 ) ;
#57610=EDGE_LOOP ( 'NONE', ( #72832, #83902 ) ) ;
#57611=CARTESIAN_POINT ( 'NONE',  ( 0.1999999999999627909, 2.500000000000000000, 0.4464101615137758272 ) ) ;
#57612=EDGE_CURVE ( 'NONE', #15438, #48671, #542, .T. ) ;
#57613=VECTOR ( 'NONE', #32567, 1000.000000000000000 ) ;
#57614=ORIENTED_EDGE ( 'NONE', *, *, #103539, .F. ) ;
#57615=ORIENTED_EDGE ( 'NONE', *, *, #25914, .T. ) ;
#57616=CARTESIAN_POINT ( 'NONE',  ( -10.80000000000000249, 2.500000000000000000, -4.230127018922197557 ) ) ;
#57617=DIRECTION ( 'NONE',  ( 0.000000000000000000, 1.000000000000000000, 0.000000000000000000 ) ) ;
#57618=FACE_BOUND ( 'NONE', #126576, .T. ) ;
#57619=DIRECTION ( 'NONE',  ( 0.000000000000000000, -0.9999939076577903929, 0.003490651415223739937 ) ) ;
#57621=CARTESIAN_POINT ( 'NONE',  ( 3.949999999999940670, 12.50000000000000000, 1.818653347947321475 ) ) ;
#57622=EDGE_CURVE ( 'NONE', #103182, #36921, #70588, .T. ) ;
#57623=AXIS2_PLACEMENT_3D ( 'NONE', #34955, #66950, #35591 ) ;
#57624=AXIS2_PLACEMENT_3D ( 'NONE', #106906, #99691, #18536 ) ;
#57625=ORIENTED_EDGE ( 'NONE', *, *, #90949, .F. ) ;
#57626=DIRECTION ( 'NONE',  ( 0.000000000000000000, 0.000000000000000000, 1.000000000000000000 ) ) ;
#57627=DIRECTION ( 'NONE',  ( 0.000000000000000000, 0.000000000000000000, 1.000000000000000000 ) ) ;
#57628=CARTESIAN_POINT ( 'NONE',  ( 9.349999999999919709, 12.50000000000000000, -6.841600689897078702 ) ) ;
#57629=DIRECTION ( 'NONE',  ( 0.000000000000000000, -0.000000000000000000, -1.000000000000000000 ) ) ;
#57630=ORIENTED_EDGE ( 'NONE', *, *, #39381, .T. ) ;
#57631=CARTESIAN_POINT ( 'NONE',  ( -3.350000000000028511, 2.500000000000000000, 2.857883832488649301 ) ) ;
#57632=FACE_OUTER_BOUND ( 'NONE', #75578, .T. ) ;
#57633=ORIENTED_EDGE ( 'NONE', *, *, #76588, .F. ) ;
#57634=ORIENTED_EDGE ( 'NONE', *, *, #39582, .F. ) ;
#57635=DIRECTION ( 'NONE',  ( 0.000000000000000000, -0.000000000000000000, 1.000000000000000000 ) ) ;
#57636=CARTESIAN_POINT ( 'NONE',  ( 13.94999999999989271, 2.500000000000000000, -1.818653347947326138 ) ) ;
#57637=VECTOR ( 'NONE', #31958, 1000.000000000000000 ) ;
#57638=FACE_BOUND ( 'NONE', #51299, .T. ) ;
#57639=CARTESIAN_POINT ( 'NONE',  ( -4.550000000000022915, 12.50000000000000000, -2.230156782645139391 ) ) ;
#57640=CIRCLE ( 'NONE', #38893, 0.1000000000000002554 ) ;
#57641=EDGE_LOOP ( 'NONE', ( #8917, #50694, #115690, #45636 ) ) ;
#57642=DIRECTION ( 'NONE',  ( 0.000000000000000000, 1.000000000000000000, 0.000000000000000000 ) ) ;
#57643=AXIS2_PLACEMENT_3D ( 'NONE', #111493, #101688, #120683 ) ;
#57644=ORIENTED_EDGE ( 'NONE', *, *, #13874, .T. ) ;
#57645=ORIENTED_EDGE ( 'NONE', *, *, #61562, .F. ) ;
#57646=DIRECTION ( 'NONE',  ( -4.274815082592931898E-19, -0.9999939076577903929, -0.003490651415223739937 ) ) ;
#57648=ORIENTED_EDGE ( 'NONE', *, *, #73601, .F. ) ;
#57649=DIRECTION ( 'NONE',  ( 0.000000000000000000, 0.000000000000000000, 1.000000000000000000 ) ) ;
#57650=DIRECTION ( 'NONE',  ( 0.000000000000000000, -0.9999939076577903929, 0.003490651415223739937 ) ) ;
#57651=AXIS2_PLACEMENT_3D ( 'NONE', #115153, #73318, #62237 ) ;
#57652=ADVANCED_FACE ( 'NONE', ( #128237 ), #6010, .T. ) ;
#57653=CIRCLE ( 'NONE', #89042, 0.1000000000000000056 ) ;
#57654=DIRECTION ( 'NONE',  ( 0.000000000000000000, 0.000000000000000000, 1.000000000000000000 ) ) ;
#57655=DIRECTION ( 'NONE',  ( 0.000000000000000000, 1.000000000000000000, 0.000000000000000000 ) ) ;
#57657=CIRCLE ( 'NONE', #107546, 0.1000000000000000472 ) ;
#57658=ADVANCED_FACE ( 'NONE', ( #98742 ), #25645, .T. ) ;
#57659=ORIENTED_EDGE ( 'NONE', *, *, #105051, .T. ) ;
#57660=AXIS2_PLACEMENT_3D ( 'NONE', #100988, #110803, #9397 ) ;
#57661=CARTESIAN_POINT ( 'NONE',  ( -3.750000000000026201, 2.500000000000000000, 5.902370205355745192 ) ) ;
#57662=CARTESIAN_POINT ( 'NONE',  ( 11.04999999999990834, 2.500000000000000000, -6.841600689897077814 ) ) ;
#57663=AXIS2_PLACEMENT_3D ( 'NONE', #112637, #30224, #62254 ) ;
#57664=DIRECTION ( 'NONE',  ( 0.000000000000000000, 0.000000000000000000, -1.000000000000000000 ) ) ;
#57665=EDGE_LOOP ( 'NONE', ( #109635, #83328 ) ) ;
#57666=ADVANCED_FACE ( 'NONE', ( #127575 ), #42389, .T. ) ;
#57667=CARTESIAN_POINT ( 'NONE',  ( -5.200000000000020606, 2.500000000000000000, -0.3464101615137782364 ) ) ;
#57668=ORIENTED_EDGE ( 'NONE', *, *, #18972, .T. ) ;
#57669=ADVANCED_FACE ( 'NONE', ( #77816 ), #107929, .T. ) ;
#57670=DIRECTION ( 'NONE',  ( 0.000000000000000000, -0.000000000000000000, 1.000000000000000000 ) ) ;
#57671=ORIENTED_EDGE ( 'NONE', *, *, #12725, .F. ) ;
#57672=FACE_OUTER_BOUND ( 'NONE', #3239, .T. ) ;
#57673=CARTESIAN_POINT ( 'NONE',  ( 17.50000000000000000, -2.499999999999999556, 3.333333333333336146 ) ) ;
#57674=CARTESIAN_POINT ( 'NONE',  ( -0.2000000000000404232, 2.500000000000000000, 3.983716857408420964 ) ) ;
#57675=CARTESIAN_POINT ( 'NONE',  ( -0.8500000000000386136, 2.500000000000000000, 1.472243186433545459 ) ) ;
#57676=ORIENTED_EDGE ( 'NONE', *, *, #6553, .T. ) ;
#57677=EDGE_CURVE ( 'NONE', #27768, #5489, #123931, .T. ) ;
#57678=CARTESIAN_POINT ( 'NONE',  ( 11.04999999999991189, 2.500000000000000000, -2.511473670974877948 ) ) ;
#57679=CARTESIAN_POINT ( 'NONE',  ( 12.69999999999990159, 12.50000000000000000, 4.741630453620009789 ) ) ;
#57681=LINE ( 'NONE', #78622, #27614 ) ;
#57682=ADVANCED_FACE ( 'NONE', ( #48368 ), #44524, .T. ) ;
#57683=AXIS2_PLACEMENT_3D ( 'NONE', #124311, #17562, #34664 ) ;
#57686=ORIENTED_EDGE ( 'NONE', *, *, #44828, .T. ) ;
#57687=DIRECTION ( 'NONE',  ( 0.000000000000000000, 0.000000000000000000, -1.000000000000000000 ) ) ;
#57688=ORIENTED_EDGE ( 'NONE', *, *, #126289, .T. ) ;
#57689=CARTESIAN_POINT ( 'NONE',  ( 3.149999999999946176, 2.500000000000000000, -1.718653347947325827 ) ) ;
#57690=ORIENTED_EDGE ( 'NONE', *, *, #55918, .T. ) ;
#57691=VERTEX_POINT ( 'NONE', #92819 ) ;
#57692=CIRCLE ( 'NONE', #80675, 0.09999999999999982514 ) ;
#57693=ORIENTED_EDGE ( 'NONE', *, *, #2418, .F. ) ;
#57694=DIRECTION ( 'NONE',  ( 0.000000000000000000, 0.000000000000000000, 1.000000000000000000 ) ) ;
#57695=AXIS2_PLACEMENT_3D ( 'NONE', #69541, #78752, #8041 ) ;
#57696=CONICAL_SURFACE ( 'NONE', #118318, 0.1000000000000000056, 0.003490658503988666988 ) ;
#57697=DIRECTION ( 'NONE',  ( 0.000000000000000000, 1.000000000000000000, 0.000000000000000000 ) ) ;
#57698=LINE ( 'NONE', #30178, #99910 ) ;
#57699=CIRCLE ( 'NONE', #84871, 0.06509327318403745899 ) ;
#57701=CARTESIAN_POINT ( 'NONE',  ( 7.499999999999923617, 2.500000000000000000, 0.5928203230275495006 ) ) ;
#57702=CARTESIAN_POINT ( 'NONE',  ( 3.549999999999940314, 12.50000000000000000, 6.841600689897072485 ) ) ;
#57703=DIRECTION ( 'NONE',  ( 0.000000000000000000, 1.000000000000000000, 0.000000000000000000 ) ) ;
#57704=DIRECTION ( 'NONE',  ( 0.000000000000000000, -0.9999939076577903929, 0.003490651415223739937 ) ) ;
#57705=ORIENTED_EDGE ( 'NONE', *, *, #75077, .T. ) ;
#57706=DIRECTION ( 'NONE',  ( 0.000000000000000000, 0.000000000000000000, 1.000000000000000000 ) ) ;
#57707=ORIENTED_EDGE ( 'NONE', *, *, #30435, .F. ) ;
#57708=VECTOR ( 'NONE', #124272, 1000.000000000000000 ) ;
#57709=EDGE_LOOP ( 'NONE', ( #16392, #99441, #63774, #119075 ) ) ;
#57710=ORIENTED_EDGE ( 'NONE', *, *, #105582, .F. ) ;
#57711=EDGE_LOOP ( 'NONE', ( #23239, #12223, #82674, #118300 ) ) ;
#57712=VECTOR ( 'NONE', #13059, 1000.000000000000000 ) ;
#57713=VECTOR ( 'NONE', #75046, 1000.000000000000000 ) ;
#57714=DIRECTION ( 'NONE',  ( 0.000000000000000000, 0.000000000000000000, -1.000000000000000000 ) ) ;
#57715=ORIENTED_EDGE ( 'NONE', *, *, #64887, .T. ) ;
#57716=ORIENTED_EDGE ( 'NONE', *, *, #78799, .T. ) ;
#57717=EDGE_CURVE ( 'NONE', #75979, #105778, #3780, .T. ) ;
#57718=DIRECTION ( 'NONE',  ( 0.000000000000000000, 0.000000000000000000, 1.000000000000000000 ) ) ;
#57719=FACE_OUTER_BOUND ( 'NONE', #121775, .T. ) ;
#57720=CIRCLE ( 'NONE', #1272, 0.06509327318403745899 ) ;
#57721=CARTESIAN_POINT ( 'NONE',  ( 4.799999999999939426, 2.500000000000000000, -4.676537180435977881 ) ) ;
#57722=DIRECTION ( 'NONE',  ( 0.000000000000000000, 0.000000000000000000, 1.000000000000000000 ) ) ;
#57723=EDGE_CURVE ( 'NONE', #53300, #1004, #77974, .T. ) ;
#57724=CARTESIAN_POINT ( 'NONE',  ( -4.550000000000026468, 2.500000000000000000, -6.595190528383302109 ) ) ;
#57725=EDGE_LOOP ( 'NONE', ( #16606, #118016 ) ) ;
#57726=ADVANCED_FACE ( 'NONE', ( #43090 ), #8913, .T. ) ;
#57727=EDGE_CURVE ( 'NONE', #4806, #24998, #121607, .T. ) ;
#57728=CARTESIAN_POINT ( 'NONE',  ( -1.050000000000038680, 12.50000000000000000, 2.511473670974873507 ) ) ;
#57729=EDGE_CURVE ( 'NONE', #107800, #48300, #100954, .T. ) ;
#57730=ORIENTED_EDGE ( 'NONE', *, *, #107661, .T. ) ;
#57731=FACE_OUTER_BOUND ( 'NONE', #127079, .T. ) ;
#57732=ORIENTED_EDGE ( 'NONE', *, *, #87960, .F. ) ;
#57733=LINE ( 'NONE', #17783, #67157 ) ;
#57734=ADVANCED_FACE ( 'NONE', ( #81689 ), #1837, .T. ) ;
#57735=EDGE_LOOP ( 'NONE', ( #87726, #50526 ) ) ;
#57736=ORIENTED_EDGE ( 'NONE', *, *, #53436, .F. ) ;
#57737=DIRECTION ( 'NONE',  ( 0.000000000000000000, -0.9999939076577903929, 0.003490651415223739937 ) ) ;
#57738=CARTESIAN_POINT ( 'NONE',  ( 3.349999999999941025, 12.50000000000000000, 7.122917578226811486 ) ) ;
#57739=EDGE_CURVE ( 'NONE', #85338, #116689, #117755, .T. ) ;
#57740=EDGE_CURVE ( 'NONE', #112785, #67757, #63346, .T. ) ;
#57742=CIRCLE ( 'NONE', #9607, 0.06509327318403745899 ) ;
#57743=DIRECTION ( 'NONE',  ( 0.000000000000000000, -0.000000000000000000, 1.000000000000000000 ) ) ;
#57744=LINE ( 'NONE', #117261, #34513 ) ;
#57745=EDGE_LOOP ( 'NONE', ( #128280, #119178 ) ) ;
#57746=CARTESIAN_POINT ( 'NONE',  ( 10.59999999999990905, 2.500000000000000000, -4.776537180435978414 ) ) ;
#57747=LINE ( 'NONE', #125810, #86985 ) ;
#57748=CARTESIAN_POINT ( 'NONE',  ( 3.149999999999946176, 2.500000000000000000, -1.818653347947325916 ) ) ;
#57749=DIRECTION ( 'NONE',  ( 0.000000000000000000, 0.000000000000000000, 1.000000000000000000 ) ) ;
#57750=CIRCLE ( 'NONE', #99792, 0.06509327318403745899 ) ;
#57751=AXIS2_PLACEMENT_3D ( 'NONE', #42348, #50240, #90127 ) ;
#57752=DIRECTION ( 'NONE',  ( 0.000000000000000000, 1.000000000000000000, 0.000000000000000000 ) ) ;
#57753=ORIENTED_EDGE ( 'NONE', *, *, #121427, .T. ) ;
#57754=VERTEX_POINT ( 'NONE', #110510 ) ;
#57755=DIRECTION ( 'NONE',  ( -0.000000000000000000, 1.000000000000000000, -0.000000000000000000 ) ) ;
#57756=VERTEX_POINT ( 'NONE', #102613 ) ;
#57757=AXIS2_PLACEMENT_3D ( 'NONE', #65614, #17795, #28278 ) ;
#57758=CONICAL_SURFACE ( 'NONE', #26457, 0.09999999999999999167, 0.003490658503988666988 ) ;
#57759=CARTESIAN_POINT ( 'NONE',  ( 12.69999999999989981, 2.500000000000000000, -0.3464101615137783474 ) ) ;
#57760=DIRECTION ( 'NONE',  ( -0.000000000000000000, 1.000000000000000000, -0.000000000000000000 ) ) ;
#57761=AXIS2_PLACEMENT_3D ( 'NONE', #3431, #82654, #72826 ) ;
#57762=VERTEX_POINT ( 'NONE', #111812 ) ;
#57764=CARTESIAN_POINT ( 'NONE',  ( 0.8499999999999536815, 12.50000000000000000, 6.560283801567334372 ) ) ;
#57765=CARTESIAN_POINT ( 'NONE',  ( -10.20000000000000462, 2.500000000000000000, 4.676537180435972552 ) ) ;
#57766=PLANE ( 'NONE',  #60172 ) ;
#57767=ORIENTED_EDGE ( 'NONE', *, *, #54538, .T. ) ;
#57768=CARTESIAN_POINT ( 'NONE',  ( -1.450000000000036371, 12.50000000000000000, 2.446380397790835826 ) ) ;
#57769=DIRECTION ( 'NONE',  ( 0.000000000000000000, 1.000000000000000000, 0.000000000000000000 ) ) ;
#57770=ORIENTED_EDGE ( 'NONE', *, *, #13825, .T. ) ;
#57771=DIRECTION ( 'NONE',  ( -0.000000000000000000, -1.000000000000000000, -0.000000000000000000 ) ) ;
#57772=AXIS2_PLACEMENT_3D ( 'NONE', #2426, #33219, #101943 ) ;
#57773=LINE ( 'NONE', #6689, #68520 ) ;
#57774=FACE_OUTER_BOUND ( 'NONE', #25903, .T. ) ;
#57775=EDGE_CURVE ( 'NONE', #3528, #47378, #71224, .T. ) ;
#57776=ORIENTED_EDGE ( 'NONE', *, *, #117775, .T. ) ;
#57777=CIRCLE ( 'NONE', #103746, 0.06509327318403745899 ) ;
#57778=DIRECTION ( 'NONE',  ( 0.000000000000000000, 0.000000000000000000, -1.000000000000000000 ) ) ;
#57779=AXIS2_PLACEMENT_3D ( 'NONE', #118351, #28701, #48995 ) ;
#57780=ORIENTED_EDGE ( 'NONE', *, *, #39476, .T. ) ;
#57781=CARTESIAN_POINT ( 'NONE',  ( 12.09999999999990195, 2.500000000000000000, -0.6928203230275541413 ) ) ;
#57782=CARTESIAN_POINT ( 'NONE',  ( -5.200000000000020606, 2.500000000000000000, 4.083716857408421497 ) ) ;
#57783=DIRECTION ( 'NONE',  ( 0.000000000000000000, 1.000000000000000000, 0.000000000000000000 ) ) ;
#57784=CONICAL_SURFACE ( 'NONE', #1334, 0.1000000000000002554, 0.003490658503988666988 ) ;
#57785=ORIENTED_EDGE ( 'NONE', *, *, #125232, .T. ) ;
#57786=DIRECTION ( 'NONE',  ( -4.274815082592931898E-19, -0.9999939076577903929, -0.003490651415223739937 ) ) ;
#57787=CONICAL_SURFACE ( 'NONE', #128912, 0.1000000000000000472, 0.003490658503988666988 ) ;
#57788=DIRECTION ( 'NONE',  ( 0.000000000000000000, 0.000000000000000000, -1.000000000000000000 ) ) ;
#57789=VERTEX_POINT ( 'NONE', #22155 ) ;
#57790=FACE_OUTER_BOUND ( 'NONE', #114409, .T. ) ;
#57791=ORIENTED_EDGE ( 'NONE', *, *, #111451, .T. ) ;
#57792=CARTESIAN_POINT ( 'NONE',  ( 14.14999999999989377, 12.50000000000000000, -1.407149913249512663 ) ) ;
#57793=CIRCLE ( 'NONE', #47427, 0.09999999999999982514 ) ;
#57794=AXIS2_PLACEMENT_3D ( 'NONE', #79741, #80400, #88924 ) ;
#57795=CIRCLE ( 'NONE', #16007, 0.06509327318403743123 ) ;
#57796=ORIENTED_EDGE ( 'NONE', *, *, #100243, .F. ) ;
#57798=PLANE ( 'NONE',  #112769 ) ;
#57799=VERTEX_POINT ( 'NONE', #50964 ) ;
#57800=ORIENTED_EDGE ( 'NONE', *, *, #70827, .F. ) ;
#57801=CARTESIAN_POINT ( 'NONE',  ( 11.89999999999990798, 12.50000000000000000, -4.676537180435977881 ) ) ;
#57802=LINE ( 'NONE', #97711, #25465 ) ;
#57803=ORIENTED_EDGE ( 'NONE', *, *, #52766, .F. ) ;
#57804=DIRECTION ( 'NONE',  ( -0.000000000000000000, -1.000000000000000000, -0.000000000000000000 ) ) ;
#57805=DIRECTION ( 'NONE',  ( 0.000000000000000000, 1.000000000000000000, 0.000000000000000000 ) ) ;
#57807=DIRECTION ( 'NONE',  ( -0.000000000000000000, -1.000000000000000000, -0.000000000000000000 ) ) ;
#57808=CARTESIAN_POINT ( 'NONE',  ( 12.89999999999990266, 2.500000000000000000, 3.637306695894644726 ) ) ;
#57809=DIRECTION ( 'NONE',  ( 0.000000000000000000, 0.000000000000000000, -1.000000000000000000 ) ) ;
#57810=EDGE_CURVE ( 'NONE', #69451, #38111, #111130, .T. ) ;
#57811=ORIENTED_EDGE ( 'NONE', *, *, #42342, .F. ) ;
#57812=ORIENTED_EDGE ( 'NONE', *, *, #37728, .T. ) ;
#57813=ORIENTED_EDGE ( 'NONE', *, *, #75242, .T. ) ;
#57814=ORIENTED_EDGE ( 'NONE', *, *, #1233, .F. ) ;
#57815=FACE_OUTER_BOUND ( 'NONE', #120021, .T. ) ;
#57816=CARTESIAN_POINT ( 'NONE',  ( -9.150000000000009237, 2.500000000000000000, -7.188010851410848723 ) ) ;
#57817=CARTESIAN_POINT ( 'NONE',  ( 3.749999999999944045, 2.500000000000000000, -2.857883832488653741 ) ) ;
#57818=ORIENTED_EDGE ( 'NONE', *, *, #69952, .F. ) ;
#57819=EDGE_CURVE ( 'NONE', #42358, #25877, #15352, .T. ) ;
#57820=FACE_BOUND ( 'NONE', #58376, .T. ) ;
#57821=ORIENTED_EDGE ( 'NONE', *, *, #102339, .T. ) ;
#57822=EDGE_CURVE ( 'NONE', #70467, #5264, #34167, .T. ) ;
#57823=DIRECTION ( 'NONE',  ( 0.000000000000000000, 1.000000000000000000, 0.000000000000000000 ) ) ;
#57824=DIRECTION ( 'NONE',  ( 0.000000000000000000, 0.000000000000000000, -1.000000000000000000 ) ) ;
#57825=DIRECTION ( 'NONE',  ( -0.000000000000000000, 1.000000000000000000, -0.000000000000000000 ) ) ;
#57826=CONICAL_SURFACE ( 'NONE', #1369, 0.1000000000000002554, 0.003490658503988666988 ) ;
#57827=CARTESIAN_POINT ( 'NONE',  ( 1.649999999999951950, 12.50000000000000000, -5.737276932171712751 ) ) ;
#57828=CONICAL_SURFACE ( 'NONE', #49425, 0.09999999999999982514, 0.003490658503988666988 ) ;
#57829=DIRECTION ( 'NONE',  ( 0.000000000000000000, -0.9999939076577903929, 0.003490651415223739937 ) ) ;
#57830=EDGE_CURVE ( 'NONE', #129204, #75499, #48746, .T. ) ;
#57831=CARTESIAN_POINT ( 'NONE',  ( -12.49999999999999467, 12.50000000000000000, -3.637306695894647390 ) ) ;
#57832=EDGE_CURVE ( 'NONE', #81547, #109936, #82188, .T. ) ;
#57833=FACE_OUTER_BOUND ( 'NONE', #110326, .T. ) ;
#57834=DIRECTION ( 'NONE',  ( 0.000000000000000000, 0.000000000000000000, 1.000000000000000000 ) ) ;
#57835=ADVANCED_FACE ( 'NONE', ( #101987 ), #52243, .T. ) ;
#57836=LINE ( 'NONE', #118670, #93652 ) ;
#57837=EDGE_CURVE ( 'NONE', #21550, #110285, #100674, .T. ) ;
#57838=EDGE_CURVE ( 'NONE', #107047, #97855, #55087, .T. ) ;
#57839=DIRECTION ( 'NONE',  ( 0.000000000000000000, 0.000000000000000000, 1.000000000000000000 ) ) ;
#57840=VECTOR ( 'NONE', #11859, 1000.000000000000000 ) ;
#57841=AXIS2_PLACEMENT_3D ( 'NONE', #59758, #118644, #86105 ) ;
#57842=ORIENTED_EDGE ( 'NONE', *, *, #53884, .T. ) ;
#57843=EDGE_LOOP ( 'NONE', ( #48190, #1073 ) ) ;
#57844=VERTEX_POINT ( 'NONE', #2469 ) ;
#57845=ORIENTED_EDGE ( 'NONE', *, *, #52733, .F. ) ;
#57846=CARTESIAN_POINT ( 'NONE',  ( -10.40000000000000213, 12.50000000000000000, -0.6928203230275541413 ) ) ;
#57847=PLANE ( 'NONE',  #77840 ) ;
#57848=ORIENTED_EDGE ( 'NONE', *, *, #75548, .T. ) ;
#57849=ORIENTED_EDGE ( 'NONE', *, *, #5778, .T. ) ;
#57850=EDGE_CURVE ( 'NONE', #124869, #35293, #12932, .T. ) ;
#57851=ORIENTED_EDGE ( 'NONE', *, *, #43401, .F. ) ;
#57852=DIRECTION ( 'NONE',  ( 0.000000000000000000, 0.000000000000000000, -1.000000000000000000 ) ) ;
#57853=CONICAL_SURFACE ( 'NONE', #45333, 0.1000000000000000472, 0.003490658503988666988 ) ;
#57854=AXIS2_PLACEMENT_3D ( 'NONE', #34782, #94979, #36057 ) ;
#57855=AXIS2_PLACEMENT_3D ( 'NONE', #102755, #33405, #63494 ) ;
#57856=PLANE ( 'NONE',  #99901 ) ;
#57857=DIRECTION ( 'NONE',  ( 0.000000000000000000, 0.000000000000000000, -1.000000000000000000 ) ) ;
#57858=DIRECTION ( 'NONE',  ( -0.000000000000000000, -1.000000000000000000, -0.000000000000000000 ) ) ;
#57859=DIRECTION ( 'NONE',  ( 0.000000000000000000, 1.000000000000000000, 0.000000000000000000 ) ) ;
#57860=DIRECTION ( 'NONE',  ( 0.000000000000000000, 0.000000000000000000, 1.000000000000000000 ) ) ;
#57861=EDGE_LOOP ( 'NONE', ( #8726, #58171, #21946, #75520 ) ) ;
#57862=LINE ( 'NONE', #109537, #49706 ) ;
#57863=EDGE_LOOP ( 'NONE', ( #66650, #105037, #61818, #46182 ) ) ;
#57864=ORIENTED_EDGE ( 'NONE', *, *, #86189, .T. ) ;
#57865=ORIENTED_EDGE ( 'NONE', *, *, #94612, .T. ) ;
#57866=DIRECTION ( 'NONE',  ( 0.000000000000000000, 0.000000000000000000, -1.000000000000000000 ) ) ;
#57867=VERTEX_POINT ( 'NONE', #115001 ) ;
#57868=CIRCLE ( 'NONE', #11869, 0.06509327318403745899 ) ;
#57869=EDGE_LOOP ( 'NONE', ( #68891, #79809, #123205, #81519 ) ) ;
#57870=CIRCLE ( 'NONE', #14212, 0.1000000000000002554 ) ;
#57872=CARTESIAN_POINT ( 'NONE',  ( -0.6500000000000389910, 2.500000000000000000, -1.818653347947326138 ) ) ;
#57873=CARTESIAN_POINT ( 'NONE',  ( 7.899999999999924860, 12.50000000000000000, 4.330127018922196314 ) ) ;
#57874=AXIS2_PLACEMENT_3D ( 'NONE', #1578, #41539, #42163 ) ;
#57875=DIRECTION ( 'NONE',  ( 0.000000000000000000, -0.9999939076577903929, 0.003490651415223739937 ) ) ;
#57876=CARTESIAN_POINT ( 'NONE',  ( -4.350000000000023626, 12.50000000000000000, 6.148780366869520897 ) ) ;
#57877=EDGE_CURVE ( 'NONE', #14270, #93574, #32123, .T. ) ;
#57878=VECTOR ( 'NONE', #63933, 1000.000000000000000 ) ;
#57879=VERTEX_POINT ( 'NONE', #116291 ) ;
#57880=ADVANCED_FACE ( 'NONE', ( #25335 ), #125480, .T. ) ;
#57881=CARTESIAN_POINT ( 'NONE',  ( 2.499999999999948930, 2.500000000000000000, -5.122947341949753763 ) ) ;
#57882=CONICAL_SURFACE ( 'NONE', #11886, 0.1000000000000002554, 0.003490658503988666988 ) ;
#57883=ORIENTED_EDGE ( 'NONE', *, *, #16981, .T. ) ;
#57884=AXIS2_PLACEMENT_3D ( 'NONE', #83202, #3975, #82562 ) ;
#57885=PLANE ( 'NONE',  #60962 ) ;
#57886=ADVANCED_FACE ( 'NONE', ( #14224 ), #128263, .T. ) ;
#57887=ORIENTED_EDGE ( 'NONE', *, *, #120084, .T. ) ;
#57888=CARTESIAN_POINT ( 'NONE',  ( 9.549999999999918998, 2.500000000000000000, 2.165063509461097713 ) ) ;
#57889=DIRECTION ( 'NONE',  ( 0.000000000000000000, 0.000000000000000000, 1.000000000000000000 ) ) ;
#57890=ORIENTED_EDGE ( 'NONE', *, *, #115148, .T. ) ;
#57891=DIRECTION ( 'NONE',  ( 0.000000000000000000, 0.000000000000000000, 1.000000000000000000 ) ) ;
#57892=CONICAL_SURFACE ( 'NONE', #5624, 0.09999999999999982514, 0.003490658503988666988 ) ;
#57893=EDGE_CURVE ( 'NONE', #47267, #30241, #103916, .T. ) ;
#57894=DIRECTION ( 'NONE',  ( -4.274815082592931898E-19, -0.9999939076577903929, -0.003490651415223739937 ) ) ;
#57895=ORIENTED_EDGE ( 'NONE', *, *, #10814, .F. ) ;
#57896=VECTOR ( 'NONE', #104153, 1000.000000000000000 ) ;
#57897=EDGE_CURVE ( 'NONE', #109253, #4262, #40440, .T. ) ;
#57898=ADVANCED_FACE ( 'NONE', ( #94093 ), #699, .T. ) ;
#57899=CIRCLE ( 'NONE', #66188, 0.1000000000000000472 ) ;
#57900=ADVANCED_FACE ( 'NONE', ( #96024 ), #107311, .T. ) ;
#57901=DIRECTION ( 'NONE',  ( 0.000000000000000000, 0.000000000000000000, 1.000000000000000000 ) ) ;
#57902=ORIENTED_EDGE ( 'NONE', *, *, #30941, .T. ) ;
#57903=VERTEX_POINT ( 'NONE', #5053 ) ;
#57904=DIRECTION ( 'NONE',  ( 0.000000000000000000, 1.000000000000000000, 0.000000000000000000 ) ) ;
#57905=CARTESIAN_POINT ( 'NONE',  ( 7.299999999999927880, 12.50000000000000000, 3.983716857408420964 ) ) ;
#57907=LINE ( 'NONE', #59857, #65852 ) ;
#57908=EDGE_CURVE ( 'NONE', #73467, #128960, #17409, .T. ) ;
#57909=DIRECTION ( 'NONE',  ( 0.000000000000000000, 1.000000000000000000, 0.000000000000000000 ) ) ;
#57910=DIRECTION ( 'NONE',  ( 0.000000000000000000, 0.000000000000000000, -1.000000000000000000 ) ) ;
#57911=AXIS2_PLACEMENT_3D ( 'NONE', #119000, #71848, #41111 ) ;
#57912=VERTEX_POINT ( 'NONE', #15516 ) ;
#57913=DIRECTION ( 'NONE',  ( 0.000000000000000000, -0.9999939076577903929, 0.003490651415223739937 ) ) ;
#57914=PLANE ( 'NONE',  #104352 ) ;
#57915=EDGE_LOOP ( 'NONE', ( #37862, #4844, #33525, #101911 ) ) ;
#57916=PLANE ( 'NONE',  #41318 ) ;
#57917=DIRECTION ( 'NONE',  ( -0.000000000000000000, 1.000000000000000000, -0.000000000000000000 ) ) ;
#57918=ADVANCED_FACE ( 'NONE', ( #115649 ), #54798, .T. ) ;
#57919=CARTESIAN_POINT ( 'NONE',  ( -7.100000000000017408, 12.50000000000000000, -4.957854068765716882 ) ) ;
#57920=FACE_OUTER_BOUND ( 'NONE', #26284, .T. ) ;
#57921=DIRECTION ( 'NONE',  ( 0.000000000000000000, 0.000000000000000000, -1.000000000000000000 ) ) ;
#57922=ORIENTED_EDGE ( 'NONE', *, *, #50184, .T. ) ;
#57923=AXIS2_PLACEMENT_3D ( 'NONE', #62107, #47449, #87350 ) ;
#57924=CARTESIAN_POINT ( 'NONE',  ( -8.950000000000009948, 2.500000000000000000, -1.918653347947326004 ) ) ;
#57925=CARTESIAN_POINT ( 'NONE',  ( -3.350000000000028955, 12.50000000000000000, -2.165063509461101710 ) ) ;
#57926=ORIENTED_EDGE ( 'NONE', *, *, #26190, .T. ) ;
#57927=CONICAL_SURFACE ( 'NONE', #80914, 0.09999999999999982514, 0.003490658503988666988 ) ;
#57928=CIRCLE ( 'NONE', #110240, 0.06509327318403745899 ) ;
#57929=DIRECTION ( 'NONE',  ( -4.274815082592931898E-19, -0.9999939076577903929, -0.003490651415223739937 ) ) ;
#57930=EDGE_CURVE ( 'NONE', #77488, #49848, #56714, .T. ) ;
#57931=VERTEX_POINT ( 'NONE', #73796 ) ;
#57932=ORIENTED_EDGE ( 'NONE', *, *, #42465, .F. ) ;
#57933=DIRECTION ( 'NONE',  ( 0.05223670945016072042, -0.9986347311133434435, 0.000000000000000000 ) ) ;
#57934=EDGE_LOOP ( 'NONE', ( #52600, #21038 ) ) ;
#57936=DIRECTION ( 'NONE',  ( 0.000000000000000000, 0.000000000000000000, 1.000000000000000000 ) ) ;
#57937=VECTOR ( 'NONE', #118909, 1000.000000000000000 ) ;
#57938=CONICAL_SURFACE ( 'NONE', #43378, 0.09999999999999982514, 0.003490658503988666988 ) ;
#57939=DIRECTION ( 'NONE',  ( 0.000000000000000000, -0.000000000000000000, 1.000000000000000000 ) ) ;
#57940=VERTEX_POINT ( 'NONE', #113744 ) ;
#57941=CONICAL_SURFACE ( 'NONE', #103906, 0.09999999999999999167, 0.003490658503988666988 ) ;
#57942=DIRECTION ( 'NONE',  ( 0.000000000000000000, 1.000000000000000000, 0.000000000000000000 ) ) ;
#57943=DIRECTION ( 'NONE',  ( 0.000000000000000000, 0.000000000000000000, 1.000000000000000000 ) ) ;
#57944=ORIENTED_EDGE ( 'NONE', *, *, #78204, .F. ) ;
#57945=DIRECTION ( 'NONE',  ( 0.000000000000000000, -0.000000000000000000, 1.000000000000000000 ) ) ;
#57946=ADVANCED_FACE ( 'NONE', ( #74454 ), #105156, .T. ) ;
#57947=CARTESIAN_POINT ( 'NONE',  ( 0.8499999999999545697, 12.50000000000000000, 2.857883832488649301 ) ) ;
#57949=ORIENTED_EDGE ( 'NONE', *, *, #8308, .F. ) ;
#57950=ORIENTED_EDGE ( 'NONE', *, *, #64956, .F. ) ;
#57951=CARTESIAN_POINT ( 'NONE',  ( -1.050000000000037348, 2.500000000000000000, -6.841600689897078702 ) ) ;
#57952=DIRECTION ( 'NONE',  ( -0.000000000000000000, -1.000000000000000000, -0.000000000000000000 ) ) ;
#57953=FACE_OUTER_BOUND ( 'NONE', #124550, .T. ) ;
#57954=FACE_BOUND ( 'NONE', #125229, .T. ) ;
#57955=ORIENTED_EDGE ( 'NONE', *, *, #24710, .T. ) ;
#57956=CIRCLE ( 'NONE', #22470, 0.1000000000000002554 ) ;
#57957=CARTESIAN_POINT ( 'NONE',  ( 1.249999999999952038, 2.500000000000000000, 5.802370205355744659 ) ) ;
#57958=DIRECTION ( 'NONE',  ( -0.000000000000000000, -1.000000000000000000, -0.000000000000000000 ) ) ;
#57959=VECTOR ( 'NONE', #60430, 1000.000000000000000 ) ;
#57960=ORIENTED_EDGE ( 'NONE', *, *, #7664, .F. ) ;
#57961=DIRECTION ( 'NONE',  ( -4.274815082592931898E-19, -0.9999939076577903929, -0.003490651415223739937 ) ) ;
#57962=AXIS2_PLACEMENT_3D ( 'NONE', #35572, #24455, #115377 ) ;
#57963=CARTESIAN_POINT ( 'NONE',  ( 5.849999999999932143, 2.500000000000000000, 2.165063509461097713 ) ) ;
#57964=CARTESIAN_POINT ( 'NONE',  ( -1.850000000000033396, 2.500000000000000000, -6.941600689897077459 ) ) ;
#57965=LINE ( 'NONE', #89355, #34726 ) ;
#57966=CARTESIAN_POINT ( 'NONE',  ( 7.299999999999927880, 12.50000000000000000, -4.676537180435977881 ) ) ;
#57967=AXIS2_PLACEMENT_3D ( 'NONE', #85503, #104494, #76334 ) ;
#57968=AXIS2_PLACEMENT_3D ( 'NONE', #118441, #38626, #106050 ) ;
#57969=EDGE_CURVE ( 'NONE', #65424, #81764, #126125, .T. ) ;
#57970=ORIENTED_EDGE ( 'NONE', *, *, #128199, .T. ) ;
#57971=ORIENTED_EDGE ( 'NONE', *, *, #96224, .T. ) ;
#57972=ORIENTED_EDGE ( 'NONE', *, *, #65789, .T. ) ;
#57973=EDGE_LOOP ( 'NONE', ( #66358, #16946, #87283, #75909 ) ) ;
#57974=ORIENTED_EDGE ( 'NONE', *, *, #83799, .T. ) ;
#57975=CARTESIAN_POINT ( 'NONE',  ( 14.79999999999989413, 12.50000000000000000, -0.3464101615137782364 ) ) ;
#57976=CARTESIAN_POINT ( 'NONE',  ( -1.900000000000035438, 2.500000000000000000, 3.983716857408420076 ) ) ;
#57978=ORIENTED_EDGE ( 'NONE', *, *, #99415, .F. ) ;
#57979=FACE_BOUND ( 'NONE', #100572, .T. ) ;
#57980=ADVANCED_FACE ( 'NONE', ( #34553 ), #92648, .T. ) ;
#57981=CARTESIAN_POINT ( 'NONE',  ( 2.499999999999947153, 2.500000000000000000, 3.637306695894644726 ) ) ;
#57982=AXIS2_PLACEMENT_3D ( 'NONE', #127260, #107606, #17931 ) ;
#57983=CIRCLE ( 'NONE', #91418, 0.06509327318403745899 ) ;
#57984=PLANE ( 'NONE',  #17801 ) ;
#57985=EDGE_CURVE ( 'NONE', #102525, #62269, #94728, .T. ) ;
#57986=CARTESIAN_POINT ( 'NONE',  ( 6.699999999999928235, 2.500000000000000000, -2.276824562219559311E-15 ) ) ;
#57987=ADVANCED_FACE ( 'NONE', ( #65257 ), #36222, .T. ) ;
#57988=PLANE ( 'NONE',  #124305 ) ;
#57989=ADVANCED_FACE ( 'NONE', ( #35817 ), #21641, .T. ) ;
#57990=DIRECTION ( 'NONE',  ( 0.000000000000000000, 1.000000000000000000, 0.000000000000000000 ) ) ;
#57991=EDGE_CURVE ( 'NONE', #99644, #73222, #38383, .T. ) ;
#57992=ORIENTED_EDGE ( 'NONE', *, *, #81200, .T. ) ;
#57993=CARTESIAN_POINT ( 'NONE',  ( 11.04999999999991189, 2.500000000000000000, 6.048780366869521252 ) ) ;
#57994=ORIENTED_EDGE ( 'NONE', *, *, #60092, .T. ) ;
#57995=ORIENTED_EDGE ( 'NONE', *, *, #75595, .F. ) ;
#57996=ORIENTED_EDGE ( 'NONE', *, *, #20241, .T. ) ;
#57997=CARTESIAN_POINT ( 'NONE',  ( 5.199999999999933564, 2.500000000000000000, 3.983716857408420076 ) ) ;
#57998=DIRECTION ( 'NONE',  ( -0.000000000000000000, 1.000000000000000000, -0.000000000000000000 ) ) ;
#57999=DIRECTION ( 'NONE',  ( 0.000000000000000000, 0.000000000000000000, 1.000000000000000000 ) ) ;
#58001=CONICAL_SURFACE ( 'NONE', #32971, 0.09999999999999982514, 0.003490658503988666988 ) ;
#58002=EDGE_CURVE ( 'NONE', #7162, #75768, #69658, .T. ) ;
#58003=CARTESIAN_POINT ( 'NONE',  ( -13.14999999999999147, 12.50000000000000000, 1.883746621131362931 ) ) ;
#58004=EDGE_CURVE ( 'NONE', #122177, #54834, #58045, .T. ) ;
#58005=DIRECTION ( 'NONE',  ( -0.000000000000000000, -1.000000000000000000, -0.000000000000000000 ) ) ;
#58006=EDGE_CURVE ( 'NONE', #102543, #29350, #52944, .T. ) ;
#58007=CARTESIAN_POINT ( 'NONE',  ( -2.700000000000030820, 2.500000000000000000, -3.983716857408426293 ) ) ;
#58009=DIRECTION ( 'NONE',  ( -0.000000000000000000, -1.000000000000000000, -0.000000000000000000 ) ) ;
#58010=PLANE ( 'NONE',  #121993 ) ;
#58011=DIRECTION ( 'NONE',  ( 0.000000000000000000, 0.000000000000000000, 1.000000000000000000 ) ) ;
#58012=ORIENTED_EDGE ( 'NONE', *, *, #82559, .F. ) ;
#58013=CARTESIAN_POINT ( 'NONE',  ( -2.500000000000032419, 12.50000000000000000, -3.702399969078687292 ) ) ;
#58014=CIRCLE ( 'NONE', #18283, 0.06509327318403745899 ) ;
#58015=ORIENTED_EDGE ( 'NONE', *, *, #34946, .T. ) ;
#58017=VERTEX_POINT ( 'NONE', #99899 ) ;
#58018=LINE ( 'NONE', #27246, #13350 ) ;
#58019=DIRECTION ( 'NONE',  ( 0.000000000000000000, -0.000000000000000000, 1.000000000000000000 ) ) ;
#58020=DIRECTION ( 'NONE',  ( 0.000000000000000000, 1.000000000000000000, 0.000000000000000000 ) ) ;
#58021=B_SPLINE_CURVE_WITH_KNOTS ( 'NONE', 3,
 ( #72800, #52499, #34166, #122545, #24340, #92428, #2754, #64252 ),
 .UNSPECIFIED., .F., .F.,
 ( 4, 2, 2, 4 ),
 ( 0.000000000000000000, 0.001904977314309959542, 0.002857465971464944084, 0.003809954628619929059 ),
 .UNSPECIFIED. ) ;
#58022=ORIENTED_EDGE ( 'NONE', *, *, #119899, .T. ) ;
#58023=AXIS2_PLACEMENT_3D ( 'NONE', #14904, #71944, #122335 ) ;
#58024=CONICAL_SURFACE ( 'NONE', #103990, 0.09999999999999982514, 0.003490658503988666988 ) ;
#58025=EDGE_LOOP ( 'NONE', ( #69262, #68972, #65726, #71350 ) ) ;
#58026=DIRECTION ( 'NONE',  ( 0.000000000000000000, 0.000000000000000000, 1.000000000000000000 ) ) ;
#58027=CIRCLE ( 'NONE', #18297, 0.06509327318403745899 ) ;
#58028=DIRECTION ( 'NONE',  ( 0.000000000000000000, 0.000000000000000000, -1.000000000000000000 ) ) ;
#58029=DIRECTION ( 'NONE',  ( -0.000000000000000000, 1.000000000000000000, -0.000000000000000000 ) ) ;
#58030=ORIENTED_EDGE ( 'NONE', *, *, #75599, .F. ) ;
#58031=EDGE_LOOP ( 'NONE', ( #99148, #75082 ) ) ;
#58032=DIRECTION ( 'NONE',  ( 0.000000000000000000, 0.000000000000000000, 1.000000000000000000 ) ) ;
#58033=AXIS2_PLACEMENT_3D ( 'NONE', #6203, #112957, #85427 ) ;
#58034=VERTEX_POINT ( 'NONE', #116935 ) ;
#58035=CARTESIAN_POINT ( 'NONE',  ( 11.24999999999994493, 12.50000000000000000, -2.099970236277064473 ) ) ;
#58036=CARTESIAN_POINT ( 'NONE',  ( -5.200000000000022382, 12.50000000000000000, 4.676537180435972552 ) ) ;
#58037=EDGE_LOOP ( 'NONE', ( #100076, #866, #112697, #9312 ) ) ;
#58038=CARTESIAN_POINT ( 'NONE',  ( 6.049999999999930544, 2.500000000000000000, 2.511473670974873507 ) ) ;
#58039=CARTESIAN_POINT ( 'NONE',  ( -12.04999999999999538, 2.500000000000000000, 2.265063509461097357 ) ) ;
#58041=EDGE_CURVE ( 'NONE', #53470, #118758, #86376, .T. ) ;
#58042=DIRECTION ( 'NONE',  ( -0.000000000000000000, -1.000000000000000000, -0.000000000000000000 ) ) ;
#58043=ORIENTED_EDGE ( 'NONE', *, *, #16829, .F. ) ;
#58044=EDGE_CURVE ( 'NONE', #67250, #122182, #29964, .T. ) ;
#58045=LINE ( 'NONE', #48213, #94796 ) ;
#58046=AXIS2_PLACEMENT_3D ( 'NONE', #45436, #23865, #46715 ) ;
#58047=B_SPLINE_CURVE_WITH_KNOTS ( 'NONE', 3,
 ( #21374, #18788, #109094, #11548 ),
 .UNSPECIFIED., .F., .F.,
 ( 4, 4 ),
 ( 0.0001556283592081808000, 0.002283789722394648485 ),
 .UNSPECIFIED. ) ;
#58048=EDGE_CURVE ( 'NONE', #53017, #18181, #6562, .T. ) ;
#58049=ORIENTED_EDGE ( 'NONE', *, *, #35822, .F. ) ;
#58050=ORIENTED_EDGE ( 'NONE', *, *, #62963, .T. ) ;
#58051=CARTESIAN_POINT ( 'NONE',  ( -2.900000000000029665, 2.500000000000000000, 4.330127018922196314 ) ) ;
#58052=DIRECTION ( 'NONE',  ( 0.000000000000000000, -0.000000000000000000, 1.000000000000000000 ) ) ;
#58053=DIRECTION ( 'NONE',  ( 0.000000000000000000, 0.000000000000000000, 1.000000000000000000 ) ) ;
#58054=CARTESIAN_POINT ( 'NONE',  ( 9.999999999999912959, 12.50000000000000000, -4.957854068765716882 ) ) ;
#58055=VECTOR ( 'NONE', #15634, 1000.000000000000000 ) ;
#58056=DIRECTION ( 'NONE',  ( 0.000000000000000000, 1.000000000000000000, 0.000000000000000000 ) ) ;
#58057=CIRCLE ( 'NONE', #112331, 0.06509327318403745899 ) ;
#58058=ADVANCED_FACE ( 'NONE', ( #88784 ), #50683, .T. ) ;
#58059=CARTESIAN_POINT ( 'NONE',  ( 5.849999999999932143, 12.50000000000000000, 1.407149913249508000 ) ) ;
#58061=CARTESIAN_POINT ( 'NONE',  ( 17.46224641143689382, 2.499999999999373834, -5.244174873149315630 ) ) ;
#58062=DIRECTION ( 'NONE',  ( -0.000000000000000000, -1.000000000000000000, -0.000000000000000000 ) ) ;
#58063=FACE_OUTER_BOUND ( 'NONE', #51571, .T. ) ;
#58064=CIRCLE ( 'NONE', #20501, 0.09999999999999982514 ) ;
#58065=CIRCLE ( 'NONE', #1604, 0.06509327318403745899 ) ;
#58066=DIRECTION ( 'NONE',  ( -0.000000000000000000, 1.000000000000000000, -0.000000000000000000 ) ) ;
#58067=ORIENTED_EDGE ( 'NONE', *, *, #5113, .F. ) ;
#58068=DIRECTION ( 'NONE',  ( 0.000000000000000000, -0.9999939076577903929, 0.003490651415223739937 ) ) ;
#58069=AXIS2_PLACEMENT_3D ( 'NONE', #58665, #98554, #27908 ) ;
#58070=PLANE ( 'NONE',  #14455 ) ;
#58071=LINE ( 'NONE', #39088, #51682 ) ;
#58072=EDGE_CURVE ( 'NONE', #126604, #11408, #80132, .T. ) ;
#58073=DIRECTION ( 'NONE',  ( 0.000000000000000000, 0.000000000000000000, 1.000000000000000000 ) ) ;
#58074=CARTESIAN_POINT ( 'NONE',  ( 13.74999999999993427, 2.500000000000000000, 2.265063509461097357 ) ) ;
#58075=ORIENTED_EDGE ( 'NONE', *, *, #40574, .F. ) ;
#58076=DIRECTION ( 'NONE',  ( 0.000000000000000000, -0.9999939076577903929, 0.003490651415223739937 ) ) ;
#58077=AXIS2_PLACEMENT_3D ( 'NONE', #3454, #72207, #21152 ) ;
#58078=CONICAL_SURFACE ( 'NONE', #74799, 0.1000000000000002554, 0.003490658503988666988 ) ;
#58079=DIRECTION ( 'NONE',  ( 0.000000000000000000, 0.000000000000000000, 1.000000000000000000 ) ) ;
#58080=DIRECTION ( 'NONE',  ( 0.000000000000000000, 1.000000000000000000, 0.000000000000000000 ) ) ;
#58081=ORIENTED_EDGE ( 'NONE', *, *, #12865, .F. ) ;
#58083=EDGE_LOOP ( 'NONE', ( #102778, #34731 ) ) ;
#58084=DIRECTION ( 'NONE',  ( -0.000000000000000000, 1.000000000000000000, -0.000000000000000000 ) ) ;
#58085=EDGE_CURVE ( 'NONE', #129486, #108759, #23793, .T. ) ;
#58086=ORIENTED_EDGE ( 'NONE', *, *, #85265, .T. ) ;
#58087=VERTEX_POINT ( 'NONE', #67848 ) ;
#58088=ORIENTED_EDGE ( 'NONE', *, *, #117794, .T. ) ;
#58089=DIRECTION ( 'NONE',  ( 0.000000000000000000, 0.000000000000000000, 1.000000000000000000 ) ) ;
#58090=CARTESIAN_POINT ( 'NONE',  ( -13.74999999999998934, 2.500000000000000000, 2.757883832488653209 ) ) ;
#58091=LINE ( 'NONE', #29916, #115232 ) ;
#58092=DIRECTION ( 'NONE',  ( 0.000000000000000000, 0.000000000000000000, 1.000000000000000000 ) ) ;
#58093=VERTEX_POINT ( 'NONE', #118889 ) ;
#58094=DIRECTION ( 'NONE',  ( 0.000000000000000000, 0.000000000000000000, 1.000000000000000000 ) ) ;
#58095=ORIENTED_EDGE ( 'NONE', *, *, #23719, .F. ) ;
#58096=DIRECTION ( 'NONE',  ( 0.000000000000000000, -0.9999939076577903929, 0.003490651415223739937 ) ) ;
#58097=FACE_OUTER_BOUND ( 'NONE', #50203, .T. ) ;
#58098=CONICAL_SURFACE ( 'NONE', #68542, 0.1000000000000000056, 0.003490658503988666988 ) ;
#58099=CARTESIAN_POINT ( 'NONE',  ( 20.25366426269097886, 2.573118374675824604, 4.179292740213257140 ) ) ;
#58101=EDGE_CURVE ( 'NONE', #66180, #997, #67689, .T. ) ;
#58102=CARTESIAN_POINT ( 'NONE',  ( 3.549999999999943867, 2.500000000000000000, -1.918653347947326004 ) ) ;
#58103=EDGE_LOOP ( 'NONE', ( #59768, #41682 ) ) ;
#58104=AXIS2_PLACEMENT_3D ( 'NONE', #34202, #65575, #13890 ) ;
#58105=AXIS2_PLACEMENT_3D ( 'NONE', #87843, #110081, #108137 ) ;
#58106=ORIENTED_EDGE ( 'NONE', *, *, #112521, .T. ) ;
#58107=ORIENTED_EDGE ( 'NONE', *, *, #101753, .T. ) ;
#58109=ORIENTED_EDGE ( 'NONE', *, *, #5843, .T. ) ;
#58110=CARTESIAN_POINT ( 'NONE',  ( 4.999999999999935163, 2.500000000000000000, 0.6928203230275494784 ) ) ;
#58111=CARTESIAN_POINT ( 'NONE',  ( -12.89999999999999147, 12.50000000000000000, 3.637306695894644726 ) ) ;
#58112=EDGE_CURVE ( 'NONE', #72972, #70798, #78337, .T. ) ;
#58113=DIRECTION ( 'NONE',  ( 0.000000000000000000, -0.000000000000000000, 1.000000000000000000 ) ) ;
#58114=FACE_BOUND ( 'NONE', #19421, .T. ) ;
#58115=DIRECTION ( 'NONE',  ( 0.000000000000000000, 1.000000000000000000, 0.000000000000000000 ) ) ;
#58117=CONICAL_SURFACE ( 'NONE', #74830, 0.09999999999999982514, 0.003490658503988666988 ) ;
#58118=PLANE ( 'NONE',  #108293 ) ;
#58119=PLANE ( 'NONE',  #129558 ) ;
#58120=AXIS2_PLACEMENT_3D ( 'NONE', #29528, #19707, #59663 ) ;
#58121=CIRCLE ( 'NONE', #95760, 0.1000000000000000472 ) ;
#58123=CARTESIAN_POINT ( 'NONE',  ( 3.549999999999944755, 12.50000000000000000, -2.511473670974877948 ) ) ;
#58124=CARTESIAN_POINT ( 'NONE',  ( 0.3999999999999628852, 12.50000000000000000, 0.7579135962115892688 ) ) ;
#58125=AXIS2_PLACEMENT_3D ( 'NONE', #104174, #46529, #98212 ) ;
#58126=FACE_OUTER_BOUND ( 'NONE', #12059, .T. ) ;
#58127=EDGE_CURVE ( 'NONE', #118142, #137, #87476, .T. ) ;
#58128=VERTEX_POINT ( 'NONE', #90056 ) ;
#58130=ORIENTED_EDGE ( 'NONE', *, *, #94195, .F. ) ;
#58131=ORIENTED_EDGE ( 'NONE', *, *, #21714, .T. ) ;
#58132=CONICAL_SURFACE ( 'NONE', #55958, 0.09999999999999982514, 0.003490658503988666988 ) ;
#58133=CARTESIAN_POINT ( 'NONE',  ( -2.700000000000029932, 2.500000000000000000, -0.3464101615137782364 ) ) ;
#58134=FACE_BOUND ( 'NONE', #52165, .T. ) ;
#58135=CARTESIAN_POINT ( 'NONE',  ( 9.349999999999916156, 2.500000000000000000, -2.511473670974877948 ) ) ;
#58136=EDGE_CURVE ( 'NONE', #96773, #85603, #84419, .T. ) ;
#58137=CONICAL_SURFACE ( 'NONE', #20482, 0.09999999999999999167, 0.003490658503988666988 ) ;
#58138=EDGE_LOOP ( 'NONE', ( #742, #75732, #123405, #73599 ) ) ;
#58139=ADVANCED_FACE ( 'NONE', ( #57393 ), #9111, .T. ) ;
#58140=DIRECTION ( 'NONE',  ( 0.000000000000000000, 0.000000000000000000, 1.000000000000000000 ) ) ;
#58141=EDGE_CURVE ( 'NONE', #84654, #109940, #109043, .T. ) ;
#58142=FACE_OUTER_BOUND ( 'NONE', #7718, .T. ) ;
#58143=ADVANCED_FACE ( 'NONE', ( #49518 ), #69754, .T. ) ;
#58144=CARTESIAN_POINT ( 'NONE',  ( -13.14999999999999147, 2.500000000000000000, 2.511473670974877503 ) ) ;
#58146=EDGE_CURVE ( 'NONE', #70759, #97670, #20056, .T. ) ;
#58147=ORIENTED_EDGE ( 'NONE', *, *, #91858, .T. ) ;
#58148=CARTESIAN_POINT ( 'NONE',  ( 10.64999999999990976, 12.50000000000000000, -6.906693963081115051 ) ) ;
#58149=AXIS2_PLACEMENT_3D ( 'NONE', #28235, #98894, #100195 ) ;
#58150=DIRECTION ( 'NONE',  ( 0.000000000000000000, 1.000000000000000000, 0.000000000000000000 ) ) ;
#58151=ORIENTED_EDGE ( 'NONE', *, *, #93477, .F. ) ;
#58152=EDGE_CURVE ( 'NONE', #85724, #63281, #61917, .T. ) ;
#58153=ORIENTED_EDGE ( 'NONE', *, *, #21602, .F. ) ;
#58154=DIRECTION ( 'NONE',  ( 0.000000000000000000, 1.000000000000000000, 0.000000000000000000 ) ) ;
#58155=EDGE_CURVE ( 'NONE', #37369, #47582, #78177, .T. ) ;
#58156=CARTESIAN_POINT ( 'NONE',  ( 12.94999999999990337, 2.500000000000000000, 2.165063509461097713 ) ) ;
#58157=CIRCLE ( 'NONE', #47490, 0.06509327318403745899 ) ;
#58158=ADVANCED_FACE ( 'NONE', ( #13429 ), #38474, .T. ) ;
#58159=EDGE_CURVE ( 'NONE', #93574, #14270, #98996, .T. ) ;
#58160=CARTESIAN_POINT ( 'NONE',  ( -7.700000000000014388, 12.50000000000000000, -4.676537180435977881 ) ) ;
#58161=ADVANCED_FACE ( 'NONE', ( #42937 ), #34268, .T. ) ;
#58162=CARTESIAN_POINT ( 'NONE',  ( -9.600000000000008527, 12.50000000000000000, 4.330127018922196314 ) ) ;
#58163=ORIENTED_EDGE ( 'NONE', *, *, #35282, .F. ) ;
#58164=DIRECTION ( 'NONE',  ( 0.000000000000000000, 1.000000000000000000, 0.000000000000000000 ) ) ;
#58165=ORIENTED_EDGE ( 'NONE', *, *, #109126, .F. ) ;
#58166=VERTEX_POINT ( 'NONE', #72382 ) ;
#58167=AXIS2_PLACEMENT_3D ( 'NONE', #116384, #27352, #8364 ) ;
#58168=EDGE_CURVE ( 'NONE', #52604, #45554, #107106, .T. ) ;
#58169=DIRECTION ( 'NONE',  ( 0.000000000000000000, 0.000000000000000000, -1.000000000000000000 ) ) ;
#58170=ADVANCED_FACE ( 'NONE', ( #30532 ), #56920, .T. ) ;
#58171=ORIENTED_EDGE ( 'NONE', *, *, #23375, .T. ) ;
#58172=DIRECTION ( 'NONE',  ( 0.000000000000000000, 0.000000000000000000, 1.000000000000000000 ) ) ;
#58173=FACE_BOUND ( 'NONE', #80796, .T. ) ;
#58174=AXIS2_PLACEMENT_3D ( 'NONE', #114683, #16471, #64300 ) ;
#58175=CIRCLE ( 'NONE', #110381, 0.06509327318403745899 ) ;
#58176=VERTEX_POINT ( 'NONE', #40997 ) ;
#58177=CARTESIAN_POINT ( 'NONE',  ( -8.350000000000013856, 2.500000000000000000, 2.165063509461097713 ) ) ;
#58178=ORIENTED_EDGE ( 'NONE', *, *, #83839, .F. ) ;
#58180=FACE_OUTER_BOUND ( 'NONE', #30666, .T. ) ;
#58181=FACE_OUTER_BOUND ( 'NONE', #41817, .T. ) ;
#58182=CARTESIAN_POINT ( 'NONE',  ( 10.84999999999991260, 12.50000000000000000, 7.122917578226811486 ) ) ;
#58183=DIRECTION ( 'NONE',  ( 0.000000000000000000, 0.000000000000000000, 1.000000000000000000 ) ) ;
#58184=EDGE_LOOP ( 'NONE', ( #15989, #4927, #20993, #62586 ) ) ;
#58185=ORIENTED_EDGE ( 'NONE', *, *, #87516, .T. ) ;
#58186=ORIENTED_EDGE ( 'NONE', *, *, #68518, .F. ) ;
#58187=DIRECTION ( 'NONE',  ( -0.000000000000000000, -1.000000000000000000, -0.000000000000000000 ) ) ;
#58188=LINE ( 'NONE', #48347, #76576 ) ;
#58189=DIRECTION ( 'NONE',  ( 0.000000000000000000, 0.000000000000000000, 1.000000000000000000 ) ) ;
#58190=VECTOR ( 'NONE', #21742, 1000.000000000000000 ) ;
#58191=VERTEX_POINT ( 'NONE', #81543 ) ;
#58192=VERTEX_POINT ( 'NONE', #40343 ) ;
#58193=ORIENTED_EDGE ( 'NONE', *, *, #9692, .F. ) ;
#58194=CARTESIAN_POINT ( 'NONE',  ( -12.49999999999995914, 2.500000000000000000, -4.230127018922199333 ) ) ;
#58195=DIRECTION ( 'NONE',  ( 0.000000000000000000, 0.000000000000000000, 1.000000000000000000 ) ) ;
#58196=VECTOR ( 'NONE', #78688, 1000.000000000000000 ) ;
#58198=DIRECTION ( 'NONE',  ( 0.000000000000000000, 1.000000000000000000, 0.000000000000000000 ) ) ;
#58199=FACE_OUTER_BOUND ( 'NONE', #49143, .T. ) ;
#58200=CONICAL_SURFACE ( 'NONE', #1728, 0.1000000000000002554, 0.003490658503988666988 ) ;
#58201=DIRECTION ( 'NONE',  ( 0.000000000000000000, 0.000000000000000000, 1.000000000000000000 ) ) ;
#58202=CARTESIAN_POINT ( 'NONE',  ( 3.749999999999978684, 12.50000000000000000, -2.099970236277064473 ) ) ;
#58205=ORIENTED_EDGE ( 'NONE', *, *, #109422, .T. ) ;
#58206=AXIS2_PLACEMENT_3D ( 'NONE', #124355, #34705, #104066 ) ;
#58207=ORIENTED_EDGE ( 'NONE', *, *, #8158, .F. ) ;
#58208=EDGE_CURVE ( 'NONE', #49054, #30916, #22638, .T. ) ;
#58209=AXIS2_PLACEMENT_3D ( 'NONE', #36471, #37106, #125469 ) ;
#58210=CARTESIAN_POINT ( 'NONE',  ( 13.14999999999990088, 12.50000000000000000, 2.511473670974873507 ) ) ;
#58211=ADVANCED_FACE ( 'NONE', ( #101828 ), #12780, .T. ) ;
#58212=DIRECTION ( 'NONE',  ( 0.000000000000000000, 0.000000000000000000, 1.000000000000000000 ) ) ;
#58213=ORIENTED_EDGE ( 'NONE', *, *, #102812, .T. ) ;
#58216=CARTESIAN_POINT ( 'NONE',  ( 2.899999999999946620, 12.50000000000000000, -0.7579135962115917113 ) ) ;
#58217=CARTESIAN_POINT ( 'NONE',  ( 8.299999999999922551, 2.500000000000000000, -4.330127018922201643 ) ) ;
#58218=CIRCLE ( 'NONE', #20551, 0.06509327318403745899 ) ;
#58219=EDGE_CURVE ( 'NONE', #47326, #129522, #119927, .T. ) ;
#58220=DIRECTION ( 'NONE',  ( 0.000000000000000000, 0.000000000000000000, 1.000000000000000000 ) ) ;
#58221=VECTOR ( 'NONE', #45185, 1000.000000000000000 ) ;
#58223=CARTESIAN_POINT ( 'NONE',  ( -5.650000000000023448, 2.500000000000000000, -2.511473670974877948 ) ) ;
#58224=DIRECTION ( 'NONE',  ( -4.274815082592931898E-19, -0.9999939076577903929, -0.003490651415223739937 ) ) ;
#58225=ORIENTED_EDGE ( 'NONE', *, *, #107633, .T. ) ;
#58226=DIRECTION ( 'NONE',  ( 0.000000000000000000, 0.000000000000000000, 1.000000000000000000 ) ) ;
#58227=CARTESIAN_POINT ( 'NONE',  ( -9.150000000000009237, 2.500000000000000000, -6.495190528383297135 ) ) ;
#58228=EDGE_LOOP ( 'NONE', ( #2002, #120578 ) ) ;
#58229=VERTEX_POINT ( 'NONE', #53381 ) ;
#58230=CIRCLE ( 'NONE', #79160, 0.06509327318403745899 ) ;
#58231=ORIENTED_EDGE ( 'NONE', *, *, #117838, .F. ) ;
#58232=EDGE_LOOP ( 'NONE', ( #10317, #87522 ) ) ;
#58234=CARTESIAN_POINT ( 'NONE',  ( -14.34999999999998543, 2.500000000000000000, 1.918653347947325338 ) ) ;
#58235=VECTOR ( 'NONE', #31339, 1000.000000000000000 ) ;
#58236=ORIENTED_EDGE ( 'NONE', *, *, #85416, .F. ) ;
#58237=CARTESIAN_POINT ( 'NONE',  ( 9.999999999999911182, 12.50000000000000000, 5.022947341949748790 ) ) ;
#58238=CARTESIAN_POINT ( 'NONE',  ( -10.20000000000000462, 12.50000000000000000, 0.4115034346978109769 ) ) ;
#58239=CARTESIAN_POINT ( 'NONE',  ( -6.250000000000021316, 12.50000000000000000, -5.802370205355749988 ) ) ;
#58240=DIRECTION ( 'NONE',  ( 0.000000000000000000, 1.000000000000000000, 0.000000000000000000 ) ) ;
#58241=EDGE_LOOP ( 'NONE', ( #39625, #79086, #39787, #73065 ) ) ;
#58242=DIRECTION ( 'NONE',  ( 0.000000000000000000, 0.000000000000000000, 1.000000000000000000 ) ) ;
#58243=CIRCLE ( 'NONE', #10110, 0.09999999999999982514 ) ;
#58244=CARTESIAN_POINT ( 'NONE',  ( -8.950000000000011724, 12.50000000000000000, -6.213873640053559022 ) ) ;
#58245=EDGE_CURVE ( 'NONE', #80023, #30581, #80229, .T. ) ;
#58246=ORIENTED_EDGE ( 'NONE', *, *, #127782, .F. ) ;
#58247=CIRCLE ( 'NONE', #8040, 0.06509327318403741736 ) ;
#58248=ORIENTED_EDGE ( 'NONE', *, *, #125068, .F. ) ;
#58249=ORIENTED_EDGE ( 'NONE', *, *, #21778, .T. ) ;
#58250=FACE_OUTER_BOUND ( 'NONE', #93906, .T. ) ;
#58251=DIRECTION ( 'NONE',  ( -0.000000000000000000, 1.000000000000000000, -0.000000000000000000 ) ) ;
#58252=EDGE_CURVE ( 'NONE', #106738, #16690, #122755, .T. ) ;
#58253=ORIENTED_EDGE ( 'NONE', *, *, #76459, .F. ) ;
#58254=CARTESIAN_POINT ( 'NONE',  ( -11.84999999999999787, 12.50000000000000000, -2.511473670974873951 ) ) ;
#58255=LINE ( 'NONE', #98153, #35005 ) ;
#58256=DIRECTION ( 'NONE',  ( 0.000000000000000000, -0.000000000000000000, 1.000000000000000000 ) ) ;
#58257=FACE_OUTER_BOUND ( 'NONE', #127725, .T. ) ;
#58258=EDGE_CURVE ( 'NONE', #115125, #74692, #493, .T. ) ;
#58260=AXIS2_PLACEMENT_3D ( 'NONE', #53315, #93234, #34974 ) ;
#58261=DIRECTION ( 'NONE',  ( 0.000000000000000000, 1.000000000000000000, 0.000000000000000000 ) ) ;
#58262=EDGE_LOOP ( 'NONE', ( #31574, #4661 ) ) ;
#58264=DIRECTION ( 'NONE',  ( -0.000000000000000000, 1.000000000000000000, -0.000000000000000000 ) ) ;
#58265=EDGE_CURVE ( 'NONE', #13639, #26682, #31171, .T. ) ;
#58266=FACE_OUTER_BOUND ( 'NONE', #73420, .T. ) ;
#58267=FACE_BOUND ( 'NONE', #106337, .T. ) ;
#58268=DIRECTION ( 'NONE',  ( 0.000000000000000000, 0.000000000000000000, 1.000000000000000000 ) ) ;
#58269=DIRECTION ( 'NONE',  ( 0.000000000000000000, -0.9999939076577903929, 0.003490651415223739937 ) ) ;
#58270=DIRECTION ( 'NONE',  ( 0.000000000000000000, 0.000000000000000000, 1.000000000000000000 ) ) ;
#58271=CONICAL_SURFACE ( 'NONE', #95828, 0.1000000000000002554, 0.003490658503988666988 ) ;
#58272=ORIENTED_EDGE ( 'NONE', *, *, #66933, .T. ) ;
#58273=DIRECTION ( 'NONE',  ( -4.274815082592931898E-19, -0.9999939076577903929, -0.003490651415223739937 ) ) ;
#58274=CARTESIAN_POINT ( 'NONE',  ( 11.44999999999991047, 12.50000000000000000, -2.511473670974877948 ) ) ;
#58275=LINE ( 'NONE', #49106, #71817 ) ;
#58277=ORIENTED_EDGE ( 'NONE', *, *, #88739, .F. ) ;
#58278=FACE_OUTER_BOUND ( 'NONE', #85378, .T. ) ;
#58279=VECTOR ( 'NONE', #88310, 1000.000000000000000 ) ;
#58280=VECTOR ( 'NONE', #16320, 1000.000000000000000 ) ;
#58281=DIRECTION ( 'NONE',  ( -0.000000000000000000, 1.000000000000000000, -0.000000000000000000 ) ) ;
#58282=AXIS2_PLACEMENT_3D ( 'NONE', #104541, #54783, #86162 ) ;
#58283=ORIENTED_EDGE ( 'NONE', *, *, #102641, .T. ) ;
#58284=EDGE_LOOP ( 'NONE', ( #1223, #117273, #65997, #48955 ) ) ;
#58285=LINE ( 'NONE', #97545, #50190 ) ;
#58286=DIRECTION ( 'NONE',  ( 0.000000000000000000, 1.000000000000000000, 0.000000000000000000 ) ) ;
#58287=FACE_BOUND ( 'NONE', #49494, .T. ) ;
#58288=CARTESIAN_POINT ( 'NONE',  ( -1.650000000000034772, 2.500000000000000000, 5.902370205355745192 ) ) ;
#58289=CIRCLE ( 'NONE', #118824, 0.1000000000000002554 ) ;
#58290=CIRCLE ( 'NONE', #112659, 0.1000000000000000472 ) ;
#58291=EDGE_CURVE ( 'NONE', #63897, #107875, #124125, .T. ) ;
#58292=VECTOR ( 'NONE', #44993, 1000.000000000000000 ) ;
#58293=VERTEX_POINT ( 'NONE', #101184 ) ;
#58294=DIRECTION ( 'NONE',  ( 0.000000000000000000, 0.000000000000000000, 1.000000000000000000 ) ) ;
#58295=ORIENTED_EDGE ( 'NONE', *, *, #92988, .F. ) ;
#58298=EDGE_CURVE ( 'NONE', #41592, #51476, #121451, .T. ) ;
#58300=AXIS2_PLACEMENT_3D ( 'NONE', #49428, #77566, #6875 ) ;
#58301=ADVANCED_FACE ( 'NONE', ( #52090 ), #103202, .T. ) ;
#58302=ORIENTED_EDGE ( 'NONE', *, *, #114460, .F. ) ;
#58303=DIRECTION ( 'NONE',  ( 0.000000000000000000, -0.9999939076577903929, 0.003490651415223739937 ) ) ;
#58305=CONICAL_SURFACE ( 'NONE', #35230, 0.1000000000000000472, 0.003490658503988666988 ) ;
#58306=EDGE_CURVE ( 'NONE', #103698, #35395, #50992, .T. ) ;
#58308=DIRECTION ( 'NONE',  ( 0.000000000000000000, -0.000000000000000000, 1.000000000000000000 ) ) ;
#58309=ADVANCED_FACE ( 'NONE', ( #73640 ), #33968, .T. ) ;
#58310=CARTESIAN_POINT ( 'NONE',  ( 6.249999999999930722, 12.50000000000000000, -1.407149913249512663 ) ) ;
#58311=AXIS2_PLACEMENT_3D ( 'NONE', #81646, #28695, #68599 ) ;
#58312=ORIENTED_EDGE ( 'NONE', *, *, #105524, .F. ) ;
#58313=DIRECTION ( 'NONE',  ( 0.000000000000000000, 0.000000000000000000, 1.000000000000000000 ) ) ;
#58314=EDGE_CURVE ( 'NONE', #106863, #2627, #90681, .T. ) ;
#58315=CARTESIAN_POINT ( 'NONE',  ( -8.950000000000009948, 12.50000000000000000, 2.576566944158910744 ) ) ;
#58316=CARTESIAN_POINT ( 'NONE',  ( 4.599999999999935696, 12.50000000000000000, 5.022947341949748790 ) ) ;
#58317=VECTOR ( 'NONE', #97334, 1000.000000000000000 ) ;
#58318=CARTESIAN_POINT ( 'NONE',  ( 21.24748442509682533, 0.7426088330904827561, -4.181982359507937730 ) ) ;
#58319=VERTEX_POINT ( 'NONE', #44849 ) ;
#58320=CARTESIAN_POINT ( 'NONE',  ( -1.050000000000038236, 12.50000000000000000, -6.213873640053564351 ) ) ;
#58321=ORIENTED_EDGE ( 'NONE', *, *, #114840, .T. ) ;
#58322=DIRECTION ( 'NONE',  ( 0.000000000000000000, 0.000000000000000000, -1.000000000000000000 ) ) ;
#58323=EDGE_CURVE ( 'NONE', #27297, #106239, #101155, .T. ) ;
#58324=ORIENTED_EDGE ( 'NONE', *, *, #12348, .F. ) ;
#58325=CARTESIAN_POINT ( 'NONE',  ( -10.40000000000000213, 12.50000000000000000, 5.022947341949748790 ) ) ;
#58326=DIRECTION ( 'NONE',  ( 0.000000000000000000, 1.000000000000000000, 0.000000000000000000 ) ) ;
#58327=PLANE ( 'NONE',  #47581 ) ;
#58328=DIRECTION ( 'NONE',  ( 0.000000000000000000, 0.000000000000000000, 1.000000000000000000 ) ) ;
#58329=EDGE_LOOP ( 'NONE', ( #65228, #1706 ) ) ;
#58330=VECTOR ( 'NONE', #90722, 1000.000000000000000 ) ;
#58331=CARTESIAN_POINT ( 'NONE',  ( 0.4499999999999573785, 12.50000000000000000, -6.430097255199264339 ) ) ;
#58332=DIRECTION ( 'NONE',  ( 0.000000000000000000, -0.9999939076577903929, 0.003490651415223739937 ) ) ;
#58333=DIRECTION ( 'NONE',  ( 0.000000000000000000, 0.000000000000000000, -1.000000000000000000 ) ) ;
#58335=FACE_OUTER_BOUND ( 'NONE', #11028, .T. ) ;
#58336=AXIS2_PLACEMENT_3D ( 'NONE', #17256, #57215, #17932 ) ;
#58337=CARTESIAN_POINT ( 'NONE',  ( 8.349999999999919709, 2.500000000000000000, 7.188010851410848723 ) ) ;
#58338=AXIS2_PLACEMENT_3D ( 'NONE', #56301, #58261, #87050 ) ;
#58339=VERTEX_POINT ( 'NONE', #14709 ) ;
#58340=VERTEX_POINT ( 'NONE', #74946 ) ;
#58341=DIRECTION ( 'NONE',  ( 0.000000000000000000, 0.000000000000000000, -1.000000000000000000 ) ) ;
#58342=EDGE_LOOP ( 'NONE', ( #87727, #111284, #85490, #129307 ) ) ;
#58343=CARTESIAN_POINT ( 'NONE',  ( -0.6500000000000398792, 12.50000000000000000, -6.906693963081115939 ) ) ;
#58344=EDGE_LOOP ( 'NONE', ( #70386, #33060 ) ) ;
#58345=EDGE_LOOP ( 'NONE', ( #16309, #100383, #110224, #112851 ) ) ;
#58347=VECTOR ( 'NONE', #72975, 1000.000000000000000 ) ;
#58348=CARTESIAN_POINT ( 'NONE',  ( 87.49999999999998579, -2.781865847474096931, -7.000342182495692178 ) ) ;
#58349=DIRECTION ( 'NONE',  ( 0.000000000000000000, -0.9999939076577903929, 0.003490651415223739937 ) ) ;
#58350=FACE_OUTER_BOUND ( 'NONE', #42631, .T. ) ;
#58351=AXIS2_PLACEMENT_3D ( 'NONE', #22337, #62259, #13120 ) ;
#58352=CIRCLE ( 'NONE', #49945, 0.1000000000000002554 ) ;
#58353=FACE_OUTER_BOUND ( 'NONE', #94244, .T. ) ;
#58354=CARTESIAN_POINT ( 'NONE',  ( 1.699999999999950218, 2.500000000000000000, 4.330127018922196314 ) ) ;
#58355=DIRECTION ( 'NONE',  ( -0.000000000000000000, -1.000000000000000000, -0.000000000000000000 ) ) ;
#58356=FACE_OUTER_BOUND ( 'NONE', #73940, .T. ) ;
#58357=AXIS2_PLACEMENT_3D ( 'NONE', #119453, #89371, #80199 ) ;
#58358=DIRECTION ( 'NONE',  ( 0.000000000000000000, 0.000000000000000000, 1.000000000000000000 ) ) ;
#58359=EDGE_LOOP ( 'NONE', ( #89414, #75549, #27740, #85996 ) ) ;
#58360=AXIS2_PLACEMENT_3D ( 'NONE', #114373, #94736, #3153 ) ;
#58361=CIRCLE ( 'NONE', #12364, 0.06509327318403745899 ) ;
#58362=EDGE_LOOP ( 'NONE', ( #123957, #29599 ) ) ;
#58363=EDGE_CURVE ( 'NONE', #52693, #23243, #44726, .T. ) ;
#58364=VERTEX_POINT ( 'NONE', #64469 ) ;
#58365=CARTESIAN_POINT ( 'NONE',  ( -3.350000000000029399, 2.500000000000000000, 6.495190528383297135 ) ) ;
#58366=ORIENTED_EDGE ( 'NONE', *, *, #9962, .T. ) ;
#58367=EDGE_LOOP ( 'NONE', ( #117104, #112069, #109473, #1302 ) ) ;
#58368=CARTESIAN_POINT ( 'NONE',  ( -9.600000000000006750, 2.500000000000000000, 0.5928203230275495006 ) ) ;
#58369=EDGE_CURVE ( 'NONE', #42274, #120872, #92748, .T. ) ;
#58370=CARTESIAN_POINT ( 'NONE',  ( -11.84999999999999787, 12.50000000000000000, -2.576566944158911188 ) ) ;
#58371=DIRECTION ( 'NONE',  ( -0.000000000000000000, -1.000000000000000000, -0.000000000000000000 ) ) ;
#58372=DIRECTION ( 'NONE',  ( 0.000000000000000000, 1.000000000000000000, 0.000000000000000000 ) ) ;
#58373=DIRECTION ( 'NONE',  ( 0.000000000000000000, -0.000000000000000000, 1.000000000000000000 ) ) ;
#58374=MANIFOLD_SOLID_BREP ( 'Boss-Extrude4', #45697 ) ;
#58375=DIRECTION ( 'NONE',  ( 0.000000000000000000, 1.000000000000000000, 0.000000000000000000 ) ) ;
#58376=EDGE_LOOP ( 'NONE', ( #61604, #83542 ) ) ;
#58377=DIRECTION ( 'NONE',  ( 0.000000000000000000, 0.000000000000000000, 1.000000000000000000 ) ) ;
#58378=EDGE_LOOP ( 'NONE', ( #96971, #8413, #112094, #99577 ) ) ;
#58379=AXIS2_PLACEMENT_3D ( 'NONE', #75134, #24103, #74491 ) ;
#58380=DIRECTION ( 'NONE',  ( -0.000000000000000000, 1.000000000000000000, -0.000000000000000000 ) ) ;
#58381=VECTOR ( 'NONE', #81702, 1000.000000000000000 ) ;
#58382=EDGE_LOOP ( 'NONE', ( #47935, #59491, #48619, #30762 ) ) ;
#58383=CARTESIAN_POINT ( 'NONE',  ( 8.549999999999922551, 2.500000000000000000, -6.148780366869526226 ) ) ;
#58384=ORIENTED_EDGE ( 'NONE', *, *, #54088, .F. ) ;
#58385=B_SPLINE_CURVE_WITH_KNOTS ( 'NONE', 3,
 ( #52537, #4069, #125145, #32924, #64918, #112110, #93118, #42750 ),
 .UNSPECIFIED., .F., .F.,
 ( 4, 2, 2, 4 ),
 ( -0.0001155885022056226470, 0.03307027595370837236, 0.04966320818166537060, 0.06625614040962236884 ),
 .UNSPECIFIED. ) ;
#58386=EDGE_LOOP ( 'NONE', ( #79191, #55361 ) ) ;
#58387=PLANE ( 'NONE',  #52375 ) ;
#58388=AXIS2_PLACEMENT_3D ( 'NONE', #37622, #55323, #77525 ) ;
#58389=CARTESIAN_POINT ( 'NONE',  ( 32.25969448929755856, -3.190781364619325267, -3.146220011503478631 ) ) ;
#58390=AXIS2_PLACEMENT_3D ( 'NONE', #97950, #76390, #107112 ) ;
#58391=AXIS2_PLACEMENT_3D ( 'NONE', #53025, #123054, #41923 ) ;
#58392=LINE ( 'NONE', #37460, #86516 ) ;
#58393=DIRECTION ( 'NONE',  ( 0.000000000000000000, 0.000000000000000000, 1.000000000000000000 ) ) ;
#58394=ORIENTED_EDGE ( 'NONE', *, *, #49867, .T. ) ;
#58395=CARTESIAN_POINT ( 'NONE',  ( 1.449999999999951328, 2.500000000000000000, 2.511473670974873507 ) ) ;
#58396=CARTESIAN_POINT ( 'NONE',  ( 4.999999999999936939, 2.500000000000000000, -0.6928203230275541413 ) ) ;
#58397=CARTESIAN_POINT ( 'NONE',  ( -9.150000000000009237, 2.500000000000000000, -6.595190528383296780 ) ) ;
#58398=CARTESIAN_POINT ( 'NONE',  ( 4.149999999999941735, 12.50000000000000000, -2.857883832488653741 ) ) ;
#58399=VECTOR ( 'NONE', #47333, 1000.000000000000000 ) ;
#58400=DIRECTION ( 'NONE',  ( -0.000000000000000000, -1.000000000000000000, -0.000000000000000000 ) ) ;
#58401=VECTOR ( 'NONE', #54202, 1000.000000000000000 ) ;
#58402=EDGE_CURVE ( 'NONE', #81742, #17997, #27683, .T. ) ;
#58403=VERTEX_POINT ( 'NONE', #85406 ) ;
#58405=CARTESIAN_POINT ( 'NONE',  ( -6.450000000000017941, 2.500000000000000000, -2.511473670974877948 ) ) ;
#58406=ORIENTED_EDGE ( 'NONE', *, *, #124593, .T. ) ;
#58407=CARTESIAN_POINT ( 'NONE',  ( -12.29999999999999716, 2.500000000000000000, 0.3464101615137776813 ) ) ;
#58408=DIRECTION ( 'NONE',  ( 0.000000000000000000, -0.000000000000000000, 1.000000000000000000 ) ) ;
#58409=EDGE_CURVE ( 'NONE', #112496, #72606, #125334, .T. ) ;
#58411=EDGE_CURVE ( 'NONE', #90074, #113119, #105049, .T. ) ;
#58412=VERTEX_POINT ( 'NONE', #61023 ) ;
#58414=FACE_OUTER_BOUND ( 'NONE', #82339, .T. ) ;
#58416=EDGE_CURVE ( 'NONE', #6453, #98508, #109263, .T. ) ;
#58417=DIRECTION ( 'NONE',  ( 0.000000000000000000, 0.000000000000000000, 1.000000000000000000 ) ) ;
#58418=EDGE_LOOP ( 'NONE', ( #99868, #22387, #36515, #119652 ) ) ;
#58419=CARTESIAN_POINT ( 'NONE',  ( 4.149999999999939959, 12.50000000000000000, -6.495190528383302464 ) ) ;
#58420=EDGE_CURVE ( 'NONE', #121861, #5978, #34065, .T. ) ;
#58421=ORIENTED_EDGE ( 'NONE', *, *, #55734, .F. ) ;
#58422=ADVANCED_FACE ( 'NONE', ( #42708 ), #2641, .T. ) ;
#58423=CARTESIAN_POINT ( 'NONE',  ( 3.749999999999938716, 2.500000000000000000, 7.288010851410849256 ) ) ;
#58424=CIRCLE ( 'NONE', #37495, 0.1000000000000002554 ) ;
#58425=DIRECTION ( 'NONE',  ( -0.000000000000000000, -1.000000000000000000, -0.000000000000000000 ) ) ;
#58426=DIRECTION ( 'NONE',  ( 0.000000000000000000, 0.000000000000000000, -1.000000000000000000 ) ) ;
#58427=ORIENTED_EDGE ( 'NONE', *, *, #67291, .T. ) ;
#58428=CARTESIAN_POINT ( 'NONE',  ( -4.150000000000024336, 2.500000000000000000, -2.065063509461102065 ) ) ;
#58429=ORIENTED_EDGE ( 'NONE', *, *, #46893, .T. ) ;
#58430=DIRECTION ( 'NONE',  ( 0.000000000000000000, 1.000000000000000000, 0.000000000000000000 ) ) ;
#58431=CONICAL_SURFACE ( 'NONE', #116887, 0.1000000000000002554, 0.003490658503988666988 ) ;
#58432=CARTESIAN_POINT ( 'NONE',  ( -8.750000000000005329, 12.50000000000000000, 5.802370205355744659 ) ) ;
#58433=FACE_OUTER_BOUND ( 'NONE', #28724, .T. ) ;
#58434=ORIENTED_EDGE ( 'NONE', *, *, #48127, .T. ) ;
#58435=DIRECTION ( 'NONE',  ( 0.000000000000000000, 1.000000000000000000, 0.000000000000000000 ) ) ;
#58436=CONICAL_SURFACE ( 'NONE', #98122, 0.1000000000000000472, 0.003490658503988666988 ) ;
#58437=CIRCLE ( 'NONE', #106446, 0.06509327318403745899 ) ;
#58440=VERTEX_POINT ( 'NONE', #80682 ) ;
#58441=CARTESIAN_POINT ( 'NONE',  ( -8.300000000000011369, 12.50000000000000000, -2.276824562219559311E-15 ) ) ;
#58442=EDGE_LOOP ( 'NONE', ( #32008, #52246 ) ) ;
#58443=FACE_OUTER_BOUND ( 'NONE', #71934, .T. ) ;
#58444=AXIS2_PLACEMENT_3D ( 'NONE', #70444, #101195, #59355 ) ;
#58445=CIRCLE ( 'NONE', #22756, 0.09999999999999999167 ) ;
#58446=EDGE_CURVE ( 'NONE', #55057, #59725, #113342, .T. ) ;
#58447=ORIENTED_EDGE ( 'NONE', *, *, #97095, .F. ) ;
#58448=DIRECTION ( 'NONE',  ( 0.000000000000000000, 0.000000000000000000, 1.000000000000000000 ) ) ;
#58449=DIRECTION ( 'NONE',  ( 0.000000000000000000, 0.000000000000000000, 1.000000000000000000 ) ) ;
#58450=ORIENTED_EDGE ( 'NONE', *, *, #98470, .F. ) ;
#58451=VERTEX_POINT ( 'NONE', #72149 ) ;
#58452=CARTESIAN_POINT ( 'NONE',  ( 9.149999999999916866, 12.50000000000000000, 5.737276932171707422 ) ) ;
#58453=FACE_OUTER_BOUND ( 'NONE', #103207, .T. ) ;
#58454=ORIENTED_EDGE ( 'NONE', *, *, #102074, .F. ) ;
#58455=ADVANCED_FACE ( 'NONE', ( #30943 ), #4689, .T. ) ;
#58456=CARTESIAN_POINT ( 'NONE',  ( -12.29999999999999716, 2.500000000000000000, -3.883716857408423984 ) ) ;
#58458=CARTESIAN_POINT ( 'NONE',  ( 9.149999999999916866, 12.50000000000000000, -2.792790559304616504 ) ) ;
#58459=FACE_OUTER_BOUND ( 'NONE', #60758, .T. ) ;
#58460=AXIS2_PLACEMENT_3D ( 'NONE', #52027, #93239, #123336 ) ;
#58461=PLANE ( 'NONE',  #82273 ) ;
#58462=EDGE_CURVE ( 'NONE', #119461, #37781, #77862, .T. ) ;
#58463=CARTESIAN_POINT ( 'NONE',  ( -11.84999999999999787, 2.500000000000000000, -2.511473670974873951 ) ) ;
#58464=DIRECTION ( 'NONE',  ( 0.000000000000000000, 0.000000000000000000, 1.000000000000000000 ) ) ;
#58465=EDGE_CURVE ( 'NONE', #34821, #83361, #75806, .T. ) ;
#58466=EDGE_CURVE ( 'NONE', #81614, #126271, #111300, .T. ) ;
#58467=AXIS2_PLACEMENT_3D ( 'NONE', #118761, #10715, #80136 ) ;
#58468=CONICAL_SURFACE ( 'NONE', #60536, 0.09999999999999982514, 0.003490658503988666988 ) ;
#58469=ORIENTED_EDGE ( 'NONE', *, *, #61409, .F. ) ;
#58470=ORIENTED_EDGE ( 'NONE', *, *, #38257, .F. ) ;
#58471=EDGE_CURVE ( 'NONE', #87106, #127915, #100846, .T. ) ;
#58472=VERTEX_POINT ( 'NONE', #100940 ) ;
#58473=ORIENTED_EDGE ( 'NONE', *, *, #95725, .T. ) ;
#58474=DIRECTION ( 'NONE',  ( -4.274815082592931898E-19, -0.9999939076577903929, -0.003490651415223739937 ) ) ;
#58475=DIRECTION ( 'NONE',  ( 0.000000000000000000, 0.000000000000000000, 1.000000000000000000 ) ) ;
#58476=DIRECTION ( 'NONE',  ( 0.000000000000000000, 1.000000000000000000, 0.000000000000000000 ) ) ;
#58477=ORIENTED_EDGE ( 'NONE', *, *, #26952, .T. ) ;
#58478=FACE_BOUND ( 'NONE', #47118, .T. ) ;
#58479=ORIENTED_EDGE ( 'NONE', *, *, #8107, .T. ) ;
#58480=CARTESIAN_POINT ( 'NONE',  ( -14.19999999999998685, 2.500000000000000000, -1.084202172485504434E-16 ) ) ;
#58481=CARTESIAN_POINT ( 'NONE',  ( -12.29999999999999538, 2.500000000000000000, -4.576537180435975571 ) ) ;
#58482=AXIS2_PLACEMENT_3D ( 'NONE', #83347, #31658, #13285 ) ;
#58483=VECTOR ( 'NONE', #54017, 1000.000000000000000 ) ;
#58484=EDGE_CURVE ( 'NONE', #111766, #82690, #92538, .T. ) ;
#58486=CIRCLE ( 'NONE', #93971, 0.1000000000000002554 ) ;
#58487=EDGE_CURVE ( 'NONE', #91091, #37483, #54880, .T. ) ;
#58488=DIRECTION ( 'NONE',  ( -0.000000000000000000, -1.000000000000000000, -0.000000000000000000 ) ) ;
#58489=DIRECTION ( 'NONE',  ( 0.000000000000000000, 1.000000000000000000, 0.000000000000000000 ) ) ;
#58491=PLANE ( 'NONE',  #106332 ) ;
#58492=CARTESIAN_POINT ( 'NONE',  ( -1.850000000000033840, 2.500000000000000000, 2.611473670974873151 ) ) ;
#58493=CARTESIAN_POINT ( 'NONE',  ( -0.6000000000000388356, 12.50000000000000000, 3.918623584224383727 ) ) ;
#58494=CIRCLE ( 'NONE', #2025, 0.09999999999999982514 ) ;
#58495=CARTESIAN_POINT ( 'NONE',  ( 4.349999999999940137, 2.500000000000000000, -6.841600689897078702 ) ) ;
#58496=VECTOR ( 'NONE', #127927, 1000.000000000000000 ) ;
#58497=VERTEX_POINT ( 'NONE', #1453 ) ;
#58498=ORIENTED_EDGE ( 'NONE', *, *, #8048, .T. ) ;
#58499=VECTOR ( 'NONE', #113464, 1000.000000000000000 ) ;
#58500=ORIENTED_EDGE ( 'NONE', *, *, #113906, .F. ) ;
#58501=ORIENTED_EDGE ( 'NONE', *, *, #39014, .F. ) ;
#58502=CARTESIAN_POINT ( 'NONE',  ( 4.999999999999973355, 2.500000000000000000, -4.330127018922201643 ) ) ;
#58503=CARTESIAN_POINT ( 'NONE',  ( -1.650000000000035216, 12.50000000000000000, -5.867463478539787225 ) ) ;
#58504=VERTEX_POINT ( 'NONE', #41408 ) ;
#58505=ORIENTED_EDGE ( 'NONE', *, *, #37481, .T. ) ;
#58506=EDGE_LOOP ( 'NONE', ( #5849, #4295 ) ) ;
#58507=PLANE ( 'NONE',  #31322 ) ;
#58508=CIRCLE ( 'NONE', #73155, 0.06509327318403745899 ) ;
#58509=DIRECTION ( 'NONE',  ( 0.000000000000000000, 0.000000000000000000, 1.000000000000000000 ) ) ;
#58510=DIRECTION ( 'NONE',  ( 0.000000000000000000, 0.000000000000000000, 1.000000000000000000 ) ) ;
#58511=DIRECTION ( 'NONE',  ( -4.274815082592931898E-19, -0.9999939076577903929, -0.003490651415223739937 ) ) ;
#58512=FACE_OUTER_BOUND ( 'NONE', #93756, .T. ) ;
#58513=AXIS2_PLACEMENT_3D ( 'NONE', #15751, #113320, #55689 ) ;
#58514=DIRECTION ( 'NONE',  ( 0.000000000000000000, 0.000000000000000000, 1.000000000000000000 ) ) ;
#58515=FACE_OUTER_BOUND ( 'NONE', #98533, .T. ) ;
#58516=VERTEX_POINT ( 'NONE', #32239 ) ;
#58517=DIRECTION ( 'NONE',  ( 0.000000000000000000, 0.000000000000000000, 1.000000000000000000 ) ) ;
#58518=EDGE_LOOP ( 'NONE', ( #85163, #128732, #38890, #88269 ) ) ;
#58519=ORIENTED_EDGE ( 'NONE', *, *, #123900, .F. ) ;
#58520=ORIENTED_EDGE ( 'NONE', *, *, #20437, .T. ) ;
#58521=CARTESIAN_POINT ( 'NONE',  ( -7.900000000000014566, 12.50000000000000000, -2.276824562219559311E-15 ) ) ;
#58522=ORIENTED_EDGE ( 'NONE', *, *, #124943, .T. ) ;
#58523=ORIENTED_EDGE ( 'NONE', *, *, #15969, .T. ) ;
#58524=DIRECTION ( 'NONE',  ( 0.000000000000000000, 1.000000000000000000, 0.000000000000000000 ) ) ;
#58525=EDGE_CURVE ( 'NONE', #120418, #93687, #23041, .T. ) ;
#58526=DIRECTION ( 'NONE',  ( -0.000000000000000000, 1.000000000000000000, -0.000000000000000000 ) ) ;
#58527=CARTESIAN_POINT ( 'NONE',  ( -2.700000000000030820, 2.500000000000000000, -3.883716857408426648 ) ) ;
#58528=CARTESIAN_POINT ( 'NONE',  ( -10.00000000000000533, 12.50000000000000000, 0.6928203230275494784 ) ) ;
#58529=DIRECTION ( 'NONE',  ( 0.000000000000000000, 1.000000000000000000, 0.000000000000000000 ) ) ;
#58530=ORIENTED_EDGE ( 'NONE', *, *, #92568, .F. ) ;
#58531=DIRECTION ( 'NONE',  ( 0.000000000000000000, 0.000000000000000000, -1.000000000000000000 ) ) ;
#58532=EDGE_LOOP ( 'NONE', ( #12419, #95135, #82796, #61007 ) ) ;
#58533=DIRECTION ( 'NONE',  ( 0.000000000000000000, 1.000000000000000000, 0.000000000000000000 ) ) ;
#58534=CIRCLE ( 'NONE', #73187, 0.06509327318403741736 ) ;
#58535=AXIS2_PLACEMENT_3D ( 'NONE', #115556, #6245, #57309 ) ;
#58536=ORIENTED_EDGE ( 'NONE', *, *, #5210, .F. ) ;
#58538=FACE_OUTER_BOUND ( 'NONE', #52370, .T. ) ;
#58539=ORIENTED_EDGE ( 'NONE', *, *, #8141, .F. ) ;
#58540=CARTESIAN_POINT ( 'NONE',  ( 11.04999999999990656, 2.500000000000000000, 2.511473670974873507 ) ) ;
#58541=CARTESIAN_POINT ( 'NONE',  ( 15.59999999999988951, 2.500000000000000000, 0.4464101615137735513 ) ) ;
#58542=ORIENTED_EDGE ( 'NONE', *, *, #89787, .T. ) ;
#58543=AXIS2_PLACEMENT_3D ( 'NONE', #5404, #27607, #45351 ) ;
#58544=CIRCLE ( 'NONE', #29289, 0.1000000000000002554 ) ;
#58545=DIRECTION ( 'NONE',  ( 0.000000000000000000, 0.000000000000000000, -1.000000000000000000 ) ) ;
#58546=EDGE_LOOP ( 'NONE', ( #113802, #90092 ) ) ;
#58547=EDGE_LOOP ( 'NONE', ( #108306, #60306, #10630, #76396 ) ) ;
#58548=DIRECTION ( 'NONE',  ( 0.000000000000000000, 0.000000000000000000, 1.000000000000000000 ) ) ;
#58549=DIRECTION ( 'NONE',  ( 0.000000000000000000, 1.000000000000000000, 0.000000000000000000 ) ) ;
#58551=FACE_OUTER_BOUND ( 'NONE', #99879, .T. ) ;
#58554=ORIENTED_EDGE ( 'NONE', *, *, #98644, .F. ) ;
#58555=DIRECTION ( 'NONE',  ( 0.000000000000000000, -0.9999939076577903929, 0.003490651415223739937 ) ) ;
#58556=AXIS2_PLACEMENT_3D ( 'NONE', #103420, #74599, #114510 ) ;
#58557=CARTESIAN_POINT ( 'NONE',  ( 8.749999999999957367, 2.500000000000000000, 2.265063509461097357 ) ) ;
#58558=EDGE_CURVE ( 'NONE', #91215, #123206, #107206, .T. ) ;
#58559=AXIS2_PLACEMENT_3D ( 'NONE', #55258, #115429, #56527 ) ;
#58560=ORIENTED_EDGE ( 'NONE', *, *, #118278, .F. ) ;
#58561=ADVANCED_FACE ( 'NONE', ( #71484 ), #61691, .T. ) ;
#58562=CARTESIAN_POINT ( 'NONE',  ( 6.849999999999929479, 2.500000000000000000, 6.741600689897071952 ) ) ;
#58563=DIRECTION ( 'NONE',  ( 0.000000000000000000, -0.9999939076577903929, 0.003490651415223739937 ) ) ;
#58564=CARTESIAN_POINT ( 'NONE',  ( -14.54999999999998472, 2.500000000000000000, -2.065063509461099844 ) ) ;
#58565=DIRECTION ( 'NONE',  ( 0.000000000000000000, 0.000000000000000000, 1.000000000000000000 ) ) ;
#58566=EDGE_CURVE ( 'NONE', #116432, #102156, #44423, .T. ) ;
#58567=CARTESIAN_POINT ( 'NONE',  ( 5.399999999999931966, 2.500000000000000000, 4.230127018922196669 ) ) ;
#58568=EDGE_LOOP ( 'NONE', ( #76627, #127642, #127510, #57970 ) ) ;
#58569=AXIS2_PLACEMENT_3D ( 'NONE', #3201, #116349, #127475 ) ;
#58570=FACE_OUTER_BOUND ( 'NONE', #18158, .T. ) ;
#58571=PLANE ( 'NONE',  #83098 ) ;
#58573=EDGE_CURVE ( 'NONE', #63390, #128977, #53151, .T. ) ;
#58574=EDGE_CURVE ( 'NONE', #96204, #83685, #52836, .T. ) ;
#58575=AXIS2_PLACEMENT_3D ( 'NONE', #60074, #109804, #48958 ) ;
#58576=EDGE_LOOP ( 'NONE', ( #31329, #25101 ) ) ;
#58577=CARTESIAN_POINT ( 'NONE',  ( 17.50000000000000000, 2.500000000000000000, -3.999999999999996447 ) ) ;
#58578=CONICAL_SURFACE ( 'NONE', #71088, 0.1000000000000002554, 0.003490658503988666988 ) ;
#58579=AXIS2_PLACEMENT_3D ( 'NONE', #21717, #72749, #41373 ) ;
#58580=EDGE_LOOP ( 'NONE', ( #47830, #128194 ) ) ;
#58581=ORIENTED_EDGE ( 'NONE', *, *, #56075, .F. ) ;
#58582=DIRECTION ( 'NONE',  ( 0.000000000000000000, 0.000000000000000000, 1.000000000000000000 ) ) ;
#58583=ORIENTED_EDGE ( 'NONE', *, *, #108766, .F. ) ;
#58584=DIRECTION ( 'NONE',  ( 0.000000000000000000, -0.000000000000000000, 1.000000000000000000 ) ) ;
#58585=DIRECTION ( 'NONE',  ( -4.274815082592931898E-19, -0.9999939076577903929, -0.003490651415223739937 ) ) ;
#58586=CIRCLE ( 'NONE', #56504, 0.06509327318403745899 ) ;
#58587=EDGE_LOOP ( 'NONE', ( #78098, #88575, #100167, #91245 ) ) ;
#58588=DIRECTION ( 'NONE',  ( 0.000000000000000000, -0.000000000000000000, 1.000000000000000000 ) ) ;
#58589=DIRECTION ( 'NONE',  ( 0.000000000000000000, 0.000000000000000000, -1.000000000000000000 ) ) ;
#58590=EDGE_LOOP ( 'NONE', ( #95059, #74950, #48129, #126866 ) ) ;
#58591=DIRECTION ( 'NONE',  ( -0.000000000000000000, -1.000000000000000000, -0.000000000000000000 ) ) ;
#58592=CARTESIAN_POINT ( 'NONE',  ( -6.650000000000015454, 2.500000000000000000, 2.957883832488649389 ) ) ;
#58593=ORIENTED_EDGE ( 'NONE', *, *, #26028, .T. ) ;
#58594=VERTEX_POINT ( 'NONE', #95008 ) ;
#58595=EDGE_LOOP ( 'NONE', ( #103281, #7105, #30910, #51157 ) ) ;
#58596=DIRECTION ( 'NONE',  ( 0.000000000000000000, -0.000000000000000000, 1.000000000000000000 ) ) ;
#58597=CARTESIAN_POINT ( 'NONE',  ( 3.749999999999978684, 2.500000000000000000, -6.395190528383301931 ) ) ;
#58598=( BOUNDED_SURFACE ( )  B_SPLINE_SURFACE ( 3, 2, ( 
 ( #74458, #3783, #62714 ),
 ( #93449, #3146, #114368 ),
 ( #31966, #54179, #53536 ),
 ( #4390, #2472, #33265 ),
 ( #101990, #51607, #71891 ),
 ( #43731, #102614, #12935 ),
 ( #91517, #12300, #63990 ),
 ( #73797, #1838, #41798 ),
 ( #52885, #84261, #33880 ),
 ( #14227, #43092, #81690 ),
 ( #73170, #83002, #52244 ),
 ( #113081, #123539, #92154 ) ),
 .UNSPECIFIED., .F., .F., .F. ) 
 B_SPLINE_SURFACE_WITH_KNOTS ( ( 4, 2, 2, 2, 2, 4 ),
 ( 3, 3 ),
 ( -5.075233897207043562E-05, 0.01652955890749042978, 0.03310987015395293331, 0.04969018140041543685, 0.05798033702364668862, 0.06627049264687794039 ),
 ( 0.000000000000000000, 1.000000000000000000 ),
 .UNSPECIFIED. ) 
 GEOMETRIC_REPRESENTATION_ITEM ( )  RATIONAL_B_SPLINE_SURFACE ( (
 ( 1.000000000000000000, 1.000000000000000000, 1.000000000000000000),
 ( 1.000000000000000000, 0.9999962913205889814, 1.000000000000000000),
 ( 1.000000000000000000, 0.9967432547768471096, 1.000000000000000000),
 ( 1.000000000000000000, 0.9780629203666471039, 1.000000000000000000),
 ( 1.000000000000000000, 0.9624374449462932413, 1.000000000000000000),
 ( 1.000000000000000000, 0.9156028756791357859, 1.000000000000000000),
 ( 1.000000000000000000, 0.8842425819005229615, 1.000000000000000000),
 ( 1.000000000000000000, 0.8293059173955059649, 1.000000000000000000),
 ( 1.000000000000000000, 0.8097380764758507210, 1.000000000000000000),
 ( 1.000000000000000000, 0.7702514575403359709, 1.000000000000000000),
 ( 1.000000000000000000, 0.7503390841289654389, 1.000000000000000000),
 ( 1.000000000000000000, 0.7318752858502187708, 1.000000000000000000) ) ) 
 REPRESENTATION_ITEM ( '' )  SURFACE ( )  );
#58599=CARTESIAN_POINT ( 'NONE',  ( 15.39999999999989022, 2.500000000000000000, -0.1000000000000023925 ) ) ;
#58600=EDGE_CURVE ( 'NONE', #84391, #85395, #85809, .T. ) ;
#58601=FACE_BOUND ( 'NONE', #108346, .T. ) ;
#58602=ORIENTED_EDGE ( 'NONE', *, *, #90615, .T. ) ;
#58603=DIRECTION ( 'NONE',  ( 0.000000000000000000, 1.000000000000000000, 0.000000000000000000 ) ) ;
#58604=CARTESIAN_POINT ( 'NONE',  ( 3.149999999999944400, 2.500000000000000000, 1.818653347947321475 ) ) ;
#58605=ORIENTED_EDGE ( 'NONE', *, *, #67880, .T. ) ;
#58607=DIRECTION ( 'NONE',  ( 0.000000000000000000, 0.000000000000000000, 1.000000000000000000 ) ) ;
#58608=AXIS2_PLACEMENT_3D ( 'NONE', #67159, #119508, #127408 ) ;
#58609=CARTESIAN_POINT ( 'NONE',  ( -6.050000000000017586, 2.500000000000000000, 1.818653347947321475 ) ) ;
#58610=EDGE_CURVE ( 'NONE', #19273, #56340, #63297, .T. ) ;
#58611=FACE_OUTER_BOUND ( 'NONE', #81349, .T. ) ;
#58612=DIRECTION ( 'NONE',  ( 0.000000000000000000, 1.000000000000000000, 0.000000000000000000 ) ) ;
#58613=EDGE_CURVE ( 'NONE', #67849, #118985, #46528, .T. ) ;
#58614=DIRECTION ( 'NONE',  ( 0.000000000000000000, 1.000000000000000000, 0.000000000000000000 ) ) ;
#58616=EDGE_CURVE ( 'NONE', #80402, #48868, #45264, .T. ) ;
#58617=AXIS2_PLACEMENT_3D ( 'NONE', #101052, #19252, #42139 ) ;
#58618=CONICAL_SURFACE ( 'NONE', #60677, 0.1000000000000002554, 0.003490658503988666988 ) ;
#58619=ORIENTED_EDGE ( 'NONE', *, *, #49201, .F. ) ;
#58620=EDGE_LOOP ( 'NONE', ( #19423, #19696 ) ) ;
#58621=EDGE_LOOP ( 'NONE', ( #52978, #115773 ) ) ;
#58622=ORIENTED_EDGE ( 'NONE', *, *, #61562, .T. ) ;
#58623=ORIENTED_EDGE ( 'NONE', *, *, #72169, .T. ) ;
#58624=DIRECTION ( 'NONE',  ( -4.274815082592931898E-19, -0.9999939076577903929, -0.003490651415223739937 ) ) ;
#58625=ADVANCED_FACE ( 'NONE', ( #66805 ), #40332, .T. ) ;
#58626=CARTESIAN_POINT ( 'NONE',  ( 7.099999999999927702, 12.50000000000000000, -3.637306695894650055 ) ) ;
#58627=EDGE_LOOP ( 'NONE', ( #19761, #7035 ) ) ;
#58628=EDGE_CURVE ( 'NONE', #102156, #116432, #59102, .T. ) ;
#58629=FACE_BOUND ( 'NONE', #93379, .T. ) ;
#58630=DIRECTION ( 'NONE',  ( 0.000000000000000000, 1.000000000000000000, 0.000000000000000000 ) ) ;
#58631=EDGE_CURVE ( 'NONE', #34514, #97550, #103000, .T. ) ;
#58632=ADVANCED_FACE ( 'NONE', ( #76650 ), #23586, .T. ) ;
#58633=ADVANCED_FACE ( 'NONE', ( #96921 ), #17399, .T. ) ;
#58634=DIRECTION ( 'NONE',  ( 0.000000000000000000, 0.000000000000000000, 1.000000000000000000 ) ) ;
#58635=DIRECTION ( 'NONE',  ( 0.000000000000000000, -0.000000000000000000, 1.000000000000000000 ) ) ;
#58636=DIRECTION ( 'NONE',  ( -0.000000000000000000, 1.000000000000000000, -0.000000000000000000 ) ) ;
#58637=CARTESIAN_POINT ( 'NONE',  ( 1.699999999999951994, 2.500000000000000000, -2.276824562219559311E-15 ) ) ;
#58638=ORIENTED_EDGE ( 'NONE', *, *, #73817, .F. ) ;
#58639=EDGE_CURVE ( 'NONE', #6619, #28229, #67476, .T. ) ;
#58640=ORIENTED_EDGE ( 'NONE', *, *, #10432, .T. ) ;
#58641=ORIENTED_EDGE ( 'NONE', *, *, #126862, .T. ) ;
#58642=ORIENTED_EDGE ( 'NONE', *, *, #117960, .F. ) ;
#58643=DIRECTION ( 'NONE',  ( 0.000000000000000000, 1.000000000000000000, 0.000000000000000000 ) ) ;
#58644=DIRECTION ( 'NONE',  ( -0.000000000000000000, 1.000000000000000000, -0.000000000000000000 ) ) ;
#58645=DIRECTION ( 'NONE',  ( -0.000000000000000000, -1.000000000000000000, -0.000000000000000000 ) ) ;
#58646=ORIENTED_EDGE ( 'NONE', *, *, #86200, .T. ) ;
#58647=DIRECTION ( 'NONE',  ( -0.000000000000000000, -1.000000000000000000, -0.000000000000000000 ) ) ;
#58648=DIRECTION ( 'NONE',  ( 0.000000000000000000, 0.000000000000000000, 1.000000000000000000 ) ) ;
#58649=CARTESIAN_POINT ( 'NONE',  ( -6.250000000000019540, 12.50000000000000000, -7.188010851410854052 ) ) ;
#58651=CARTESIAN_POINT ( 'NONE',  ( 10.59999999999991260, 2.500000000000000000, -0.3464101615137783474 ) ) ;
#58652=DIRECTION ( 'NONE',  ( 0.000000000000000000, 0.000000000000000000, -1.000000000000000000 ) ) ;
#58653=DIRECTION ( 'NONE',  ( 0.000000000000000000, 0.000000000000000000, 1.000000000000000000 ) ) ;
#58654=VERTEX_POINT ( 'NONE', #94341 ) ;
#58655=DIRECTION ( 'NONE',  ( -0.000000000000000000, 1.000000000000000000, -0.000000000000000000 ) ) ;
#58656=CONICAL_SURFACE ( 'NONE', #106748, 0.1000000000000002554, 0.003490658503988666988 ) ;
#58657=ORIENTED_EDGE ( 'NONE', *, *, #99975, .T. ) ;
#58658=EDGE_LOOP ( 'NONE', ( #39750, #93485 ) ) ;
#58659=CARTESIAN_POINT ( 'NONE',  ( -5.850000000000019185, 12.50000000000000000, 2.165063509461097713 ) ) ;
#58660=DIRECTION ( 'NONE',  ( 0.000000000000000000, 1.000000000000000000, 0.000000000000000000 ) ) ;
#58661=CARTESIAN_POINT ( 'NONE',  ( -8.350000000000013856, 2.500000000000000000, -6.395190528383296602 ) ) ;
#58662=VERTEX_POINT ( 'NONE', #5953 ) ;
#58663=ORIENTED_EDGE ( 'NONE', *, *, #82565, .F. ) ;
#58664=AXIS2_PLACEMENT_3D ( 'NONE', #126981, #96860, #124405 ) ;
#58665=CARTESIAN_POINT ( 'NONE',  ( 12.29999999999990479, 2.500000000000000000, -3.983716857408426293 ) ) ;
#58666=AXIS2_PLACEMENT_3D ( 'NONE', #38806, #12993, #83061 ) ;
#58667=EDGE_CURVE ( 'NONE', #93997, #27988, #67578, .T. ) ;
#58668=CARTESIAN_POINT ( 'NONE',  ( -8.749999999999971578, 12.50000000000000000, 6.560283801567334372 ) ) ;
#58669=CARTESIAN_POINT ( 'NONE',  ( 2.500000000000002220, -1.500000000000000000, -9.999999999999998224 ) ) ;
#58670=ORIENTED_EDGE ( 'NONE', *, *, #105991, .T. ) ;
#58671=ORIENTED_EDGE ( 'NONE', *, *, #25300, .T. ) ;
#58672=LINE ( 'NONE', #69119, #64845 ) ;
#58673=VECTOR ( 'NONE', #106547, 1000.000000000000000 ) ;
#58674=ORIENTED_EDGE ( 'NONE', *, *, #58002, .F. ) ;
#58675=DIRECTION ( 'NONE',  ( -0.000000000000000000, -1.000000000000000000, -0.000000000000000000 ) ) ;
#58676=ORIENTED_EDGE ( 'NONE', *, *, #55513, .T. ) ;
#58677=DIRECTION ( 'NONE',  ( 0.000000000000000000, 0.000000000000000000, 1.000000000000000000 ) ) ;
#58678=LINE ( 'NONE', #48871, #46236 ) ;
#58679=AXIS2_PLACEMENT_3D ( 'NONE', #111215, #119768, #22877 ) ;
#58680=CARTESIAN_POINT ( 'NONE',  ( 3.149999999999942624, 2.500000000000000000, 6.741600689897071952 ) ) ;
#58681=ADVANCED_FACE ( 'NONE', ( #26267 ), #15245, .T. ) ;
#58682=DIRECTION ( 'NONE',  ( 0.000000000000000000, 1.000000000000000000, 0.000000000000000000 ) ) ;
#58684=DIRECTION ( 'NONE',  ( 0.000000000000000000, 0.000000000000000000, 1.000000000000000000 ) ) ;
#58685=EDGE_LOOP ( 'NONE', ( #7576, #28448 ) ) ;
#58686=ORIENTED_EDGE ( 'NONE', *, *, #103650, .T. ) ;
#58687=CARTESIAN_POINT ( 'NONE',  ( -1.700000000000035261, 2.500000000000000000, 4.430127018922196847 ) ) ;
#58688=DIRECTION ( 'NONE',  ( 0.000000000000000000, 0.000000000000000000, 1.000000000000000000 ) ) ;
#58689=DIRECTION ( 'NONE',  ( 0.000000000000000000, 0.000000000000000000, 1.000000000000000000 ) ) ;
#58690=DIRECTION ( 'NONE',  ( 0.000000000000000000, 0.000000000000000000, 1.000000000000000000 ) ) ;
#58691=CARTESIAN_POINT ( 'NONE',  ( 0.6499999999999543920, 12.50000000000000000, 6.213873640053559022 ) ) ;
#58692=CARTESIAN_POINT ( 'NONE',  ( -7.300000000000016698, 2.500000000000000000, -0.3464101615137783474 ) ) ;
#58693=FACE_OUTER_BOUND ( 'NONE', #66537, .T. ) ;
#58694=CARTESIAN_POINT ( 'NONE',  ( -8.750000000000007105, 2.500000000000000000, 7.188010851410848723 ) ) ;
#58695=DIRECTION ( 'NONE',  ( 0.000000000000000000, 1.000000000000000000, 0.000000000000000000 ) ) ;
#58696=AXIS2_PLACEMENT_3D ( 'NONE', #81219, #78654, #109380 ) ;
#58697=AXIS2_PLACEMENT_3D ( 'NONE', #46607, #123869, #96338 ) ;
#58698=CIRCLE ( 'NONE', #46164, 0.06509327318403745899 ) ;
#58699=CARTESIAN_POINT ( 'NONE',  ( 0.6499999999999566125, 12.50000000000000000, -6.841600689897077814 ) ) ;
#58700=EDGE_CURVE ( 'NONE', #43111, #112381, #111395, .T. ) ;
#58701=CIRCLE ( 'NONE', #18973, 0.06509327318403745899 ) ;
#58702=ORIENTED_EDGE ( 'NONE', *, *, #8004, .F. ) ;
#58703=DIRECTION ( 'NONE',  ( 0.000000000000000000, -0.9999939076577903929, 0.003490651415223739937 ) ) ;
#58704=AXIS2_PLACEMENT_3D ( 'NONE', #1019, #1654, #110331 ) ;
#58705=CARTESIAN_POINT ( 'NONE',  ( -5.800000000000018474, 2.500000000000000000, -0.1000000000000022815 ) ) ;
#58706=DIRECTION ( 'NONE',  ( 0.000000000000000000, 0.000000000000000000, -1.000000000000000000 ) ) ;
#58707=DIRECTION ( 'NONE',  ( -0.000000000000000000, 1.000000000000000000, -0.000000000000000000 ) ) ;
#58708=CARTESIAN_POINT ( 'NONE',  ( 3.749999999999942268, 2.500000000000000000, 1.472243186433545459 ) ) ;
#58709=EDGE_CURVE ( 'NONE', #38624, #60290, #121876, .T. ) ;
#58710=ORIENTED_EDGE ( 'NONE', *, *, #74741, .T. ) ;
#58711=FACE_OUTER_BOUND ( 'NONE', #33992, .T. ) ;
#58713=CARTESIAN_POINT ( 'NONE',  ( -1.650000000000035216, 2.500000000000000000, -1.572243186433550211 ) ) ;
#58714=VERTEX_POINT ( 'NONE', #104795 ) ;
#58715=ADVANCED_FACE ( 'NONE', ( #114004 ), #125103, .T. ) ;
#58716=ADVANCED_FACE ( 'NONE', ( #65532 ), #107302, .T. ) ;
#58717=EDGE_CURVE ( 'NONE', #65306, #83794, #27885, .T. ) ;
#58718=ADVANCED_FACE ( 'NONE', ( #8527 ), #49784, .T. ) ;
#58719=ADVANCED_FACE ( 'NONE', ( #89689 ), #65439, .T. ) ;
#58720=ORIENTED_EDGE ( 'NONE', *, *, #59383, .T. ) ;
#58721=DIRECTION ( 'NONE',  ( -0.000000000000000000, 1.000000000000000000, -0.000000000000000000 ) ) ;
#58722=EDGE_LOOP ( 'NONE', ( #90146, #72939 ) ) ;
#58723=ORIENTED_EDGE ( 'NONE', *, *, #25578, .F. ) ;
#58724=VERTEX_POINT ( 'NONE', #9840 ) ;
#58725=FACE_OUTER_BOUND ( 'NONE', #117788, .T. ) ;
#58726=EDGE_CURVE ( 'NONE', #55549, #77652, #8998, .T. ) ;
#58727=DIRECTION ( 'NONE',  ( 0.000000000000000000, 0.000000000000000000, 1.000000000000000000 ) ) ;
#58728=DIRECTION ( 'NONE',  ( 0.000000000000000000, 1.000000000000000000, 0.000000000000000000 ) ) ;
#58729=EDGE_CURVE ( 'NONE', #6508, #20003, #100937, .T. ) ;
#58730=CARTESIAN_POINT ( 'NONE',  ( 10.39999999999991154, 2.500000000000000000, -4.922947341949753586 ) ) ;
#58731=ADVANCED_FACE ( 'NONE', ( #108679 ), #105145, .T. ) ;
#58732=ORIENTED_EDGE ( 'NONE', *, *, #115500, .T. ) ;
#58733=AXIS2_PLACEMENT_3D ( 'NONE', #56708, #77020, #7622 ) ;
#58734=CARTESIAN_POINT ( 'NONE',  ( 1.049999999999953637, 2.500000000000000000, 2.511473670974873507 ) ) ;
#58735=ORIENTED_EDGE ( 'NONE', *, *, #38037, .F. ) ;
#58736=CARTESIAN_POINT ( 'NONE',  ( -5.200000000000020606, 2.500000000000000000, 3.983716857408420964 ) ) ;
#58737=CARTESIAN_POINT ( 'NONE',  ( 18.78720903127623032, -2.539625591034306407, -4.564429507521173157 ) ) ;
#58738=CARTESIAN_POINT ( 'NONE',  ( 2.949999999999946887, 2.500000000000000000, -2.165063509461101710 ) ) ;
#58739=DIRECTION ( 'NONE',  ( 0.000000000000000000, -0.000000000000000000, 1.000000000000000000 ) ) ;
#58740=DIRECTION ( 'NONE',  ( 0.000000000000000000, 0.000000000000000000, 1.000000000000000000 ) ) ;
#58741=AXIS2_PLACEMENT_3D ( 'NONE', #50004, #2813, #21156 ) ;
#58742=ORIENTED_EDGE ( 'NONE', *, *, #77191, .T. ) ;
#58743=AXIS2_PLACEMENT_3D ( 'NONE', #102149, #93611, #81841 ) ;
#58744=ORIENTED_EDGE ( 'NONE', *, *, #34546, .T. ) ;
#58745=EDGE_LOOP ( 'NONE', ( #82089, #61269 ) ) ;
#58746=ORIENTED_EDGE ( 'NONE', *, *, #34363, .T. ) ;
#58748=CARTESIAN_POINT ( 'NONE',  ( 8.149999999999923972, 2.500000000000000000, -6.248780366869526759 ) ) ;
#58749=CARTESIAN_POINT ( 'NONE',  ( 65.39894234688509300, 3.129862333795020657, 5.811320850201310506 ) ) ;
#58750=CARTESIAN_POINT ( 'NONE',  ( -13.74999999999995381, 12.50000000000000000, -2.165063509461099489 ) ) ;
#58751=FACE_BOUND ( 'NONE', #77797, .T. ) ;
#58752=DIRECTION ( 'NONE',  ( 0.000000000000000000, 1.000000000000000000, 0.000000000000000000 ) ) ;
#58754=CARTESIAN_POINT ( 'NONE',  ( 9.999999999999914735, 2.500000000000000000, 0.7928203230275495672 ) ) ;
#58755=DIRECTION ( 'NONE',  ( 0.000000000000000000, 1.000000000000000000, 0.000000000000000000 ) ) ;
#58756=CONICAL_SURFACE ( 'NONE', #98442, 0.1000000000000002554, 0.003490658503988666988 ) ;
#58757=CIRCLE ( 'NONE', #2296, 0.06509327318403745899 ) ;
#58759=CARTESIAN_POINT ( 'NONE',  ( -7.950000000000016165, 12.50000000000000000, -6.495190528383297135 ) ) ;
#58760=DIRECTION ( 'NONE',  ( 0.000000000000000000, 1.000000000000000000, 0.000000000000000000 ) ) ;
#58761=CIRCLE ( 'NONE', #127799, 0.09999999999999982514 ) ;
#58762=CARTESIAN_POINT ( 'NONE',  ( 5.849999999999932143, 12.50000000000000000, 2.230156782645134950 ) ) ;
#58763=ADVANCED_FACE ( 'NONE', ( #127048 ), #113570, .T. ) ;
#58764=ORIENTED_EDGE ( 'NONE', *, *, #22365, .T. ) ;
#58765=CIRCLE ( 'NONE', #127713, 0.1000000000000000472 ) ;
#58766=VERTEX_POINT ( 'NONE', #39955 ) ;
#58767=VERTEX_POINT ( 'NONE', #119792 ) ;
#58768=ORIENTED_EDGE ( 'NONE', *, *, #65633, .F. ) ;
#58769=CARTESIAN_POINT ( 'NONE',  ( -6.450000000000014388, 12.50000000000000000, 1.753560074763284016 ) ) ;
#58770=DIRECTION ( 'NONE',  ( 0.000000000000000000, -0.000000000000000000, 1.000000000000000000 ) ) ;
#58771=EDGE_CURVE ( 'NONE', #21419, #69282, #71708, .T. ) ;
#58772=FACE_BOUND ( 'NONE', #83129, .T. ) ;
#58773=CARTESIAN_POINT ( 'NONE',  ( 10.84999999999991260, 2.500000000000000000, 7.288010851410849256 ) ) ;
#58774=EDGE_CURVE ( 'NONE', #70218, #120216, #29952, .T. ) ;
#58775=EDGE_CURVE ( 'NONE', #7138, #54276, #88421, .T. ) ;
#58776=EDGE_LOOP ( 'NONE', ( #41531, #103595 ) ) ;
#58777=CARTESIAN_POINT ( 'NONE',  ( -6.650000000000018119, 2.500000000000000000, -2.165063509461101710 ) ) ;
#58778=LINE ( 'NONE', #14471, #59956 ) ;
#58779=LINE ( 'NONE', #91295, #62484 ) ;
#58780=CARTESIAN_POINT ( 'NONE',  ( -5.600000000000020073, 2.500000000000000000, 0.3464101615137736845 ) ) ;
#58781=ORIENTED_EDGE ( 'NONE', *, *, #67117, .T. ) ;
#58783=ADVANCED_FACE ( 'NONE', ( #38683 ), #77965, .T. ) ;
#58785=VERTEX_POINT ( 'NONE', #47846 ) ;
#58786=AXIS2_PLACEMENT_3D ( 'NONE', #75253, #24869, #64782 ) ;
#58787=VERTEX_POINT ( 'NONE', #87738 ) ;
#58788=PLANE ( 'NONE',  #6864 ) ;
#58790=PLANE ( 'NONE',  #20427 ) ;
#58791=ORIENTED_EDGE ( 'NONE', *, *, #43954, .T. ) ;
#58792=DIRECTION ( 'NONE',  ( 0.000000000000000000, 0.000000000000000000, 1.000000000000000000 ) ) ;
#58793=CONICAL_SURFACE ( 'NONE', #16975, 0.09999999999999999167, 0.003490658503988666988 ) ;
#58794=CARTESIAN_POINT ( 'NONE',  ( -6.050000000000020250, 2.500000000000000000, -6.841600689897078702 ) ) ;
#58795=AXIS2_PLACEMENT_3D ( 'NONE', #34517, #45618, #124813 ) ;
#58796=ORIENTED_EDGE ( 'NONE', *, *, #126748, .F. ) ;
#58797=DIRECTION ( 'NONE',  ( 0.000000000000000000, 1.000000000000000000, 0.000000000000000000 ) ) ;
#58798=ORIENTED_EDGE ( 'NONE', *, *, #45238, .T. ) ;
#58799=CIRCLE ( 'NONE', #60938, 0.06509327318403743123 ) ;
#58800=CARTESIAN_POINT ( 'NONE',  ( -6.900000000000019007, 12.50000000000000000, -3.918623584224389056 ) ) ;
#58801=EDGE_CURVE ( 'NONE', #74701, #72217, #115606, .T. ) ;
#58802=EDGE_LOOP ( 'NONE', ( #89406, #111108, #83641, #32312 ) ) ;
#58803=CARTESIAN_POINT ( 'NONE',  ( 0.1999999999999567124, 2.500000000000000000, -3.983716857408426293 ) ) ;
#58804=FACE_BOUND ( 'NONE', #57610, .T. ) ;
#58805=ORIENTED_EDGE ( 'NONE', *, *, #73086, .T. ) ;
#58806=CARTESIAN_POINT ( 'NONE',  ( -2.900000000000029665, 2.500000000000000000, 3.637306695894644726 ) ) ;
#58807=ORIENTED_EDGE ( 'NONE', *, *, #49861, .T. ) ;
#58808=DIRECTION ( 'NONE',  ( 0.000000000000000000, -0.9999939076577903929, 0.003490651415223739937 ) ) ;
#58809=DIRECTION ( 'NONE',  ( 0.000000000000000000, 0.000000000000000000, 1.000000000000000000 ) ) ;
#58811=CARTESIAN_POINT ( 'NONE',  ( 3.749999999999940492, 2.500000000000000000, 5.702370205355745014 ) ) ;
#58812=FACE_OUTER_BOUND ( 'NONE', #32688, .T. ) ;
#58813=ORIENTED_EDGE ( 'NONE', *, *, #35114, .T. ) ;
#58814=ORIENTED_EDGE ( 'NONE', *, *, #90285, .T. ) ;
#58815=EDGE_LOOP ( 'NONE', ( #70085, #31198, #90003, #18449 ) ) ;
#58816=DIRECTION ( 'NONE',  ( -0.000000000000000000, -1.000000000000000000, -0.000000000000000000 ) ) ;
#58817=EDGE_CURVE ( 'NONE', #128968, #96874, #73854, .T. ) ;
#58818=CARTESIAN_POINT ( 'NONE',  ( -9.800000000000006040, 12.50000000000000000, 0.4115034346978109769 ) ) ;
#58819=LINE ( 'NONE', #98724, #56442 ) ;
#58820=ORIENTED_EDGE ( 'NONE', *, *, #97604, .T. ) ;
#58821=VERTEX_POINT ( 'NONE', #122176 ) ;
#58822=ORIENTED_EDGE ( 'NONE', *, *, #97529, .T. ) ;
#58823=PLANE ( 'NONE',  #49882 ) ;
#58824=AXIS2_PLACEMENT_3D ( 'NONE', #47606, #88129, #105873 ) ;
#58825=DIRECTION ( 'NONE',  ( -0.000000000000000000, -1.000000000000000000, -0.000000000000000000 ) ) ;
#58826=AXIS2_PLACEMENT_3D ( 'NONE', #106954, #96483, #17268 ) ;
#58827=DIRECTION ( 'NONE',  ( 0.000000000000000000, 1.000000000000000000, 0.000000000000000000 ) ) ;
#58828=CARTESIAN_POINT ( 'NONE',  ( -6.850000000000017408, 2.500000000000000000, -6.841600689897077814 ) ) ;
#58829=CARTESIAN_POINT ( 'NONE',  ( 11.44999999999990692, 12.50000000000000000, 1.818653347947321475 ) ) ;
#58830=CARTESIAN_POINT ( 'NONE',  ( 4.349999999999938360, 12.50000000000000000, 1.753560074763284016 ) ) ;
#58831=LINE ( 'NONE', #89577, #75944 ) ;
#58832=EDGE_CURVE ( 'NONE', #87563, #103647, #2738, .T. ) ;
#58833=CARTESIAN_POINT ( 'NONE',  ( -6.650000000000014566, 12.50000000000000000, 5.867463478539781896 ) ) ;
#58834=ORIENTED_EDGE ( 'NONE', *, *, #117199, .F. ) ;
#58835=AXIS2_PLACEMENT_3D ( 'NONE', #69960, #129547, #9744 ) ;
#58836=ORIENTED_EDGE ( 'NONE', *, *, #48973, .T. ) ;
#58837=DIRECTION ( 'NONE',  ( 0.000000000000000000, 1.000000000000000000, 0.000000000000000000 ) ) ;
#58838=DIRECTION ( 'NONE',  ( 0.000000000000000000, -0.000000000000000000, 1.000000000000000000 ) ) ;
#58839=EDGE_LOOP ( 'NONE', ( #121265, #24016 ) ) ;
#58840=VERTEX_POINT ( 'NONE', #103170 ) ;
#58842=DIRECTION ( 'NONE',  ( 0.000000000000000000, 0.000000000000000000, -1.000000000000000000 ) ) ;
#58843=LINE ( 'NONE', #128899, #107272 ) ;
#58844=FACE_OUTER_BOUND ( 'NONE', #24663, .T. ) ;
#58846=AXIS2_PLACEMENT_3D ( 'NONE', #87386, #27826, #98491 ) ;
#58847=DIRECTION ( 'NONE',  ( -0.000000000000000000, 1.000000000000000000, -0.000000000000000000 ) ) ;
#58848=LINE ( 'NONE', #555, #7187 ) ;
#58849=VECTOR ( 'NONE', #90746, 1000.000000000000000 ) ;
#58850=DIRECTION ( 'NONE',  ( 0.000000000000000000, 0.000000000000000000, -1.000000000000000000 ) ) ;
#58851=VECTOR ( 'NONE', #48132, 1000.000000000000000 ) ;
#58852=DIRECTION ( 'NONE',  ( 0.000000000000000000, 0.000000000000000000, -1.000000000000000000 ) ) ;
#58853=ORIENTED_EDGE ( 'NONE', *, *, #25632, .F. ) ;
#58854=EDGE_CURVE ( 'NONE', #96136, #80214, #13195, .T. ) ;
#58855=CIRCLE ( 'NONE', #37924, 0.1000000000000000056 ) ;
#58856=AXIS2_PLACEMENT_3D ( 'NONE', #87470, #26001, #27268 ) ;
#58857=VERTEX_POINT ( 'NONE', #12193 ) ;
#58858=ORIENTED_EDGE ( 'NONE', *, *, #91688, .F. ) ;
#58859=ORIENTED_EDGE ( 'NONE', *, *, #79152, .T. ) ;
#58860=DIRECTION ( 'NONE',  ( 0.000000000000000000, -0.9999939076577903929, 0.003490651415223739937 ) ) ;
#58861=FACE_OUTER_BOUND ( 'NONE', #101855, .T. ) ;
#58863=ORIENTED_EDGE ( 'NONE', *, *, #123486, .T. ) ;
#58864=DIRECTION ( 'NONE',  ( 0.000000000000000000, 0.000000000000000000, 1.000000000000000000 ) ) ;
#58865=CARTESIAN_POINT ( 'NONE',  ( 17.50000000000000000, -0.9166666666666696273, -2.864912725862979848 ) ) ;
#58869=ADVANCED_FACE ( 'NONE', ( #72430 ), #3045, .T. ) ;
#58870=EDGE_CURVE ( 'NONE', #50389, #64315, #119827, .T. ) ;
#58871=EDGE_CURVE ( 'NONE', #40542, #23039, #13482, .T. ) ;
#58872=DIRECTION ( 'NONE',  ( 0.000000000000000000, 1.000000000000000000, 0.000000000000000000 ) ) ;
#58873=EDGE_CURVE ( 'NONE', #79801, #59178, #80123, .T. ) ;
#58874=CARTESIAN_POINT ( 'NONE',  ( 1.849999999999950573, 12.50000000000000000, -1.818653347947326138 ) ) ;
#58875=EDGE_LOOP ( 'NONE', ( #103475, #731, #63336, #69933 ) ) ;
#58876=ORIENTED_EDGE ( 'NONE', *, *, #123033, .F. ) ;
#58877=EDGE_CURVE ( 'NONE', #89429, #3071, #40429, .T. ) ;
#58878=ORIENTED_EDGE ( 'NONE', *, *, #91850, .T. ) ;
#58879=CIRCLE ( 'NONE', #109026, 0.06509327318403745899 ) ;
#58880=ORIENTED_EDGE ( 'NONE', *, *, #43518, .F. ) ;
#58881=DIRECTION ( 'NONE',  ( -0.000000000000000000, 1.000000000000000000, -0.000000000000000000 ) ) ;
#58882=CIRCLE ( 'NONE', #127824, 0.1000000000000000472 ) ;
#58883=CIRCLE ( 'NONE', #75587, 0.06509327318403745899 ) ;
#58884=ADVANCED_FACE ( 'NONE', ( #111703 ), #71125, .T. ) ;
#58885=EDGE_CURVE ( 'NONE', #35899, #106061, #93352, .T. ) ;
#58886=CARTESIAN_POINT ( 'NONE',  ( 14.99999999999992895, 12.50000000000000000, -2.276824562219559311E-15 ) ) ;
#58887=ADVANCED_FACE ( 'NONE', ( #111029 ), #86453, .T. ) ;
#58888=AXIS2_PLACEMENT_3D ( 'NONE', #78549, #90260, #9141 ) ;
#58889=EDGE_CURVE ( 'NONE', #104132, #37082, #101885, .T. ) ;
#58890=AXIS2_PLACEMENT_3D ( 'NONE', #120783, #21965, #51427 ) ;
#58891=CONICAL_SURFACE ( 'NONE', #2430, 0.1000000000000002554, 0.003490658503988666988 ) ;
#58892=ORIENTED_EDGE ( 'NONE', *, *, #57622, .F. ) ;
#58893=CARTESIAN_POINT ( 'NONE',  ( -8.150000000000009237, 2.500000000000000000, 6.941600689897073018 ) ) ;
#58894=CARTESIAN_POINT ( 'NONE',  ( 19.52519901027828197, -0.5909487300084618200, -4.333354523369954414 ) ) ;
#58895=DIRECTION ( 'NONE',  ( 0.000000000000000000, 1.000000000000000000, 0.000000000000000000 ) ) ;
#58896=CARTESIAN_POINT ( 'NONE',  ( 5.849999999999932143, 2.500000000000000000, 2.165063509461097713 ) ) ;
#58897=EDGE_CURVE ( 'NONE', #18181, #82263, #107888, .T. ) ;
#58898=VECTOR ( 'NONE', #27208, 1000.000000000000000 ) ;
#58899=EDGE_LOOP ( 'NONE', ( #96319, #56818 ) ) ;
#58900=CARTESIAN_POINT ( 'NONE',  ( -2.100000000000034728, 12.50000000000000000, 4.395220292106234439 ) ) ;
#58901=ORIENTED_EDGE ( 'NONE', *, *, #8713, .T. ) ;
#58902=ORIENTED_EDGE ( 'NONE', *, *, #112585, .F. ) ;
#58903=LINE ( 'NONE', #17670, #112400 ) ;
#58904=DIRECTION ( 'NONE',  ( 0.000000000000000000, 0.000000000000000000, 1.000000000000000000 ) ) ;
#58905=FACE_BOUND ( 'NONE', #76286, .T. ) ;
#58906=DIRECTION ( 'NONE',  ( -0.000000000000000000, 1.000000000000000000, -0.000000000000000000 ) ) ;
#58907=DIRECTION ( 'NONE',  ( 0.000000000000000000, 0.000000000000000000, -1.000000000000000000 ) ) ;
#58908=DIRECTION ( 'NONE',  ( 0.000000000000000000, 0.000000000000000000, 1.000000000000000000 ) ) ;
#58909=ORIENTED_EDGE ( 'NONE', *, *, #30554, .T. ) ;
#58910=DIRECTION ( 'NONE',  ( 0.000000000000000000, 1.000000000000000000, 0.000000000000000000 ) ) ;
#58911=CARTESIAN_POINT ( 'NONE',  ( -11.89999999999999680, 2.500000000000000000, -3.883716857408423984 ) ) ;
#58912=DIRECTION ( 'NONE',  ( 0.000000000000000000, 0.000000000000000000, 1.000000000000000000 ) ) ;
#58913=DIRECTION ( 'NONE',  ( -0.000000000000000000, 1.000000000000000000, -0.000000000000000000 ) ) ;
#58914=VERTEX_POINT ( 'NONE', #105083 ) ;
#58915=CIRCLE ( 'NONE', #23297, 0.06509327318403745899 ) ;
#58916=CARTESIAN_POINT ( 'NONE',  ( 2.699999999999946443, 2.500000000000000000, -3.983716857408426293 ) ) ;
#58917=CARTESIAN_POINT ( 'NONE',  ( 9.999999999999911182, 2.500000000000000000, -3.537306695894649966 ) ) ;
#58918=VERTEX_POINT ( 'NONE', #94625 ) ;
#58919=ORIENTED_EDGE ( 'NONE', *, *, #69687, .T. ) ;
#58920=CARTESIAN_POINT ( 'NONE',  ( -3.150000000000030109, 2.500000000000000000, -2.611473670974877592 ) ) ;
#58921=CARTESIAN_POINT ( 'NONE',  ( -3.300000000000028244, 2.500000000000000000, 4.230127018922196669 ) ) ;
#58922=FACE_BOUND ( 'NONE', #125770, .T. ) ;
#58924=CARTESIAN_POINT ( 'NONE',  ( -14.34999999999998543, 2.500000000000000000, 1.718653347947325383 ) ) ;
#58925=AXIS2_PLACEMENT_3D ( 'NONE', #93276, #74926, #124017 ) ;
#58926=EDGE_CURVE ( 'NONE', #54395, #35289, #16694, .T. ) ;
#58927=VERTEX_POINT ( 'NONE', #15413 ) ;
#58928=AXIS2_PLACEMENT_3D ( 'NONE', #122147, #23271, #103132 ) ;
#58929=DIRECTION ( 'NONE',  ( 0.000000000000000000, 0.000000000000000000, -1.000000000000000000 ) ) ;
#58930=VECTOR ( 'NONE', #112087, 1000.000000000000000 ) ;
#58931=ADVANCED_FACE ( 'NONE', ( #95924 ), #44610, .T. ) ;
#58932=VERTEX_POINT ( 'NONE', #14756 ) ;
#58933=LINE ( 'NONE', #49128, #8957 ) ;
#58935=ORIENTED_EDGE ( 'NONE', *, *, #111194, .F. ) ;
#58936=VECTOR ( 'NONE', #127952, 1000.000000000000000 ) ;
#58937=PLANE ( 'NONE',  #126339 ) ;
#58938=CARTESIAN_POINT ( 'NONE',  ( 8.949999999999919353, 12.50000000000000000, 2.511473670974873507 ) ) ;
#58939=EDGE_CURVE ( 'NONE', #45959, #119467, #23786, .T. ) ;
#58940=AXIS2_PLACEMENT_3D ( 'NONE', #3531, #75481, #34943 ) ;
#58941=EDGE_CURVE ( 'NONE', #61697, #41126, #107391, .T. ) ;
#58942=AXIS2_PLACEMENT_3D ( 'NONE', #78081, #59753, #68248 ) ;
#58943=AXIS2_PLACEMENT_3D ( 'NONE', #42092, #204, #40159 ) ;
#58944=AXIS2_PLACEMENT_3D ( 'NONE', #18696, #58643, #98530 ) ;
#58945=DIRECTION ( 'NONE',  ( -0.000000000000000000, 1.000000000000000000, -0.000000000000000000 ) ) ;
#58946=CARTESIAN_POINT ( 'NONE',  ( 11.24999999999990585, 2.500000000000000000, 2.757883832488649656 ) ) ;
#58947=CIRCLE ( 'NONE', #2488, 0.1000000000000002554 ) ;
#58948=ORIENTED_EDGE ( 'NONE', *, *, #36154, .F. ) ;
#58950=CIRCLE ( 'NONE', #67319, 0.09999999999999982514 ) ;
#58951=DIRECTION ( 'NONE',  ( 0.000000000000000000, 1.000000000000000000, 0.000000000000000000 ) ) ;
#58952=LINE ( 'NONE', #68107, #91032 ) ;
#58953=LINE ( 'NONE', #28849, #51186 ) ;
#58954=VERTEX_POINT ( 'NONE', #93995 ) ;
#58955=EDGE_LOOP ( 'NONE', ( #77531, #89624, #80590, #92604 ) ) ;
#58956=EDGE_LOOP ( 'NONE', ( #91902, #106095, #102406, #119863 ) ) ;
#58958=CARTESIAN_POINT ( 'NONE',  ( 87.50000000000001421, -3.974992050023845369, 6.359987280038161828 ) ) ;
#58959=CARTESIAN_POINT ( 'NONE',  ( -0.8500000000000386136, 2.500000000000000000, 1.472243186433545459 ) ) ;
#58960=CARTESIAN_POINT ( 'NONE',  ( -12.69999999999999041, 12.50000000000000000, 3.983716857408420964 ) ) ;
#58961=VERTEX_POINT ( 'NONE', #6231 ) ;
#58962=FACE_OUTER_BOUND ( 'NONE', #25057, .T. ) ;
#58963=CARTESIAN_POINT ( 'NONE',  ( -9.150000000000009237, 2.500000000000000000, -2.757883832488654097 ) ) ;
#58964=DIRECTION ( 'NONE',  ( 0.000000000000000000, 0.000000000000000000, 1.000000000000000000 ) ) ;
#58966=CARTESIAN_POINT ( 'NONE',  ( 0.5999999999999551248, 2.500000000000000000, -4.576537180435978236 ) ) ;
#58967=DIRECTION ( 'NONE',  ( 0.000000000000000000, -0.9999939076577903929, 0.003490651415223739937 ) ) ;
#58968=EDGE_CURVE ( 'NONE', #98422, #34323, #24615, .T. ) ;
#58969=ORIENTED_EDGE ( 'NONE', *, *, #40005, .T. ) ;
#58970=EDGE_LOOP ( 'NONE', ( #71834, #60622 ) ) ;
#58971=CARTESIAN_POINT ( 'NONE',  ( 8.349999999999923261, 2.500000000000000000, 1.572243186433545548 ) ) ;
#58972=VERTEX_POINT ( 'NONE', #103820 ) ;
#58973=CIRCLE ( 'NONE', #94552, 0.09999999999999982514 ) ;
#58974=CARTESIAN_POINT ( 'NONE',  ( 15.19999999999989093, 2.500000000000000000, 0.2464101615137735679 ) ) ;
#58975=CIRCLE ( 'NONE', #119592, 0.06509327318403745899 ) ;
#58976=ORIENTED_EDGE ( 'NONE', *, *, #124170, .T. ) ;
#58977=VERTEX_POINT ( 'NONE', #126016 ) ;
#58978=EDGE_LOOP ( 'NONE', ( #129540, #31686, #118287, #76701 ) ) ;
#58979=CARTESIAN_POINT ( 'NONE',  ( 17.50000000000000000, -0.4166666666666616337, -3.999999999999996447 ) ) ;
#58980=FACE_OUTER_BOUND ( 'NONE', #86765, .T. ) ;
#58981=CONICAL_SURFACE ( 'NONE', #50657, 0.09999999999999999167, 0.003490658503988666988 ) ;
#58982=CIRCLE ( 'NONE', #31793, 0.09999999999999982514 ) ;
#58983=LINE ( 'NONE', #48, #91488 ) ;
#58984=CIRCLE ( 'NONE', #79807, 0.09999999999999982514 ) ;
#58985=DIRECTION ( 'NONE',  ( -0.000000000000000000, -1.000000000000000000, -0.000000000000000000 ) ) ;
#58986=DIRECTION ( 'NONE',  ( -0.000000000000000000, 1.000000000000000000, -0.000000000000000000 ) ) ;
#58987=AXIS2_PLACEMENT_3D ( 'NONE', #37565, #108218, #106290 ) ;
#58988=EDGE_CURVE ( 'NONE', #109829, #10701, #61340, .T. ) ;
#58990=DIRECTION ( 'NONE',  ( -0.000000000000000000, -1.000000000000000000, -0.000000000000000000 ) ) ;
#58991=AXIS2_PLACEMENT_3D ( 'NONE', #74823, #7351, #15889 ) ;
#58993=FACE_OUTER_BOUND ( 'NONE', #82901, .T. ) ;
#58994=EDGE_LOOP ( 'NONE', ( #53110, #73529, #126941, #72999 ) ) ;
#58995=VERTEX_POINT ( 'NONE', #84809 ) ;
#58996=FACE_OUTER_BOUND ( 'NONE', #129574, .T. ) ;
#58997=ORIENTED_EDGE ( 'NONE', *, *, #128067, .T. ) ;
#58998=EDGE_CURVE ( 'NONE', #49639, #48345, #50984, .T. ) ;
#58999=ORIENTED_EDGE ( 'NONE', *, *, #48952, .T. ) ;
#59000=LINE ( 'NONE', #68813, #100544 ) ;
#59001=PLANE ( 'NONE',  #100580 ) ;
#59002=LINE ( 'NONE', #108087, #121655 ) ;
#59003=CARTESIAN_POINT ( 'NONE',  ( 5.199999999999931788, 2.500000000000000000, 4.676537180435972552 ) ) ;
#59004=DIRECTION ( 'NONE',  ( -0.000000000000000000, -1.000000000000000000, -0.000000000000000000 ) ) ;
#59005=ORIENTED_EDGE ( 'NONE', *, *, #10516, .F. ) ;
#59006=AXIS2_PLACEMENT_3D ( 'NONE', #27295, #98602, #67193 ) ;
#59007=VERTEX_POINT ( 'NONE', #66457 ) ;
#59008=DIRECTION ( 'NONE',  ( -0.000000000000000000, -1.000000000000000000, -0.000000000000000000 ) ) ;
#59009=ORIENTED_EDGE ( 'NONE', *, *, #106270, .F. ) ;
#59010=DIRECTION ( 'NONE',  ( 0.000000000000000000, 1.000000000000000000, 0.000000000000000000 ) ) ;
#59011=ORIENTED_EDGE ( 'NONE', *, *, #42508, .F. ) ;
#59012=ORIENTED_EDGE ( 'NONE', *, *, #114252, .F. ) ;
#59013=AXIS2_PLACEMENT_3D ( 'NONE', #65148, #35090, #76287 ) ;
#59014=CARTESIAN_POINT ( 'NONE',  ( 8.349999999999923261, 2.500000000000000000, 1.572243186433545548 ) ) ;
#59015=PLANE ( 'NONE',  #54797 ) ;
#59016=AXIS2_PLACEMENT_3D ( 'NONE', #49355, #58524, #68317 ) ;
#59017=AXIS2_PLACEMENT_3D ( 'NONE', #121962, #121311, #32319 ) ;
#59018=ADVANCED_FACE ( 'NONE', ( #4291 ), #2845, .T. ) ;
#59019=FACE_OUTER_BOUND ( 'NONE', #78267, .T. ) ;
#59020=AXIS2_PLACEMENT_3D ( 'NONE', #124059, #74963, #94584 ) ;
#59021=DIRECTION ( 'NONE',  ( 0.000000000000000000, 1.000000000000000000, 0.000000000000000000 ) ) ;
#59022=CARTESIAN_POINT ( 'NONE',  ( 12.69999999999990159, 2.500000000000000000, -3.983716857408426293 ) ) ;
#59023=ORIENTED_EDGE ( 'NONE', *, *, #108837, .T. ) ;
#59024=CARTESIAN_POINT ( 'NONE',  ( 12.89999999999990266, 12.50000000000000000, 4.957854068765711553 ) ) ;
#59025=CARTESIAN_POINT ( 'NONE',  ( -0.8000000000000381251, 12.50000000000000000, 4.330127018922196314 ) ) ;
#59026=EDGE_CURVE ( 'NONE', #60686, #104656, #17494, .T. ) ;
#59027=CARTESIAN_POINT ( 'NONE',  ( 2.949999999999943334, 12.50000000000000000, 6.560283801567334372 ) ) ;
#59028=ADVANCED_FACE ( 'NONE', ( #54069 ), #40526, .T. ) ;
#59029=DIRECTION ( 'NONE',  ( 0.000000000000000000, 0.000000000000000000, -1.000000000000000000 ) ) ;
#59030=EDGE_CURVE ( 'NONE', #120803, #120419, #67677, .T. ) ;
#59031=AXIS2_PLACEMENT_3D ( 'NONE', #80152, #114582, #20586 ) ;
#59032=CONICAL_SURFACE ( 'NONE', #13028, 0.1000000000000000472, 0.003490658503988666988 ) ;
#59033=LINE ( 'NONE', #68190, #66761 ) ;
#59034=VERTEX_POINT ( 'NONE', #75620 ) ;
#59035=AXIS2_PLACEMENT_3D ( 'NONE', #55099, #106129, #14506 ) ;
#59036=VERTEX_POINT ( 'NONE', #84161 ) ;
#59038=CARTESIAN_POINT ( 'NONE',  ( -10.85000000000000142, 2.500000000000000000, -6.395190528383298378 ) ) ;
#59039=EDGE_CURVE ( 'NONE', #88979, #62189, #124094, .T. ) ;
#59040=AXIS2_PLACEMENT_3D ( 'NONE', #29465, #69370, #89670 ) ;
#59041=EDGE_LOOP ( 'NONE', ( #40432, #45684 ) ) ;
#59042=CARTESIAN_POINT ( 'NONE',  ( -5.200000000000020606, 2.500000000000000000, 3.983716857408420964 ) ) ;
#59043=CARTESIAN_POINT ( 'NONE',  ( -11.64999999999999858, 2.500000000000000000, -1.472243186433546125 ) ) ;
#59044=ADVANCED_FACE ( 'NONE', ( #34446 ), #27977, .T. ) ;
#59045=CIRCLE ( 'NONE', #104989, 0.1000000000000000472 ) ;
#59046=ORIENTED_EDGE ( 'NONE', *, *, #51653, .F. ) ;
#59047=DIRECTION ( 'NONE',  ( 0.000000000000000000, 1.000000000000000000, 0.000000000000000000 ) ) ;
#59048=DIRECTION ( 'NONE',  ( 0.000000000000000000, 0.000000000000000000, -1.000000000000000000 ) ) ;
#59049=EDGE_CURVE ( 'NONE', #121438, #99874, #25901, .T. ) ;
#59050=DIRECTION ( 'NONE',  ( -0.000000000000000000, 1.000000000000000000, -0.000000000000000000 ) ) ;
#59051=FACE_OUTER_BOUND ( 'NONE', #92802, .T. ) ;
#59052=ORIENTED_EDGE ( 'NONE', *, *, #71720, .T. ) ;
#59053=ADVANCED_FACE ( 'NONE', ( #78884 ), #108317, .T. ) ;
#59054=LINE ( 'NONE', #98972, #116707 ) ;
#59055=VERTEX_POINT ( 'NONE', #48124 ) ;
#59056=AXIS2_PLACEMENT_3D ( 'NONE', #19067, #126477, #87173 ) ;
#59057=CARTESIAN_POINT ( 'NONE',  ( 7.299999999999926104, 12.50000000000000000, 4.611443907251934426 ) ) ;
#59058=CARTESIAN_POINT ( 'NONE',  ( -0.4500000000000402012, 12.50000000000000000, 6.560283801567334372 ) ) ;
#59059=DIRECTION ( 'NONE',  ( 0.000000000000000000, 1.000000000000000000, 0.000000000000000000 ) ) ;
#59060=ORIENTED_EDGE ( 'NONE', *, *, #69786, .T. ) ;
#59061=CARTESIAN_POINT ( 'NONE',  ( -5.400000000000020783, 2.500000000000000000, 5.122947341949749323 ) ) ;
#59062=AXIS2_PLACEMENT_3D ( 'NONE', #58609, #79533, #78904 ) ;
#59063=CIRCLE ( 'NONE', #63258, 0.06509327318403745899 ) ;
#59064=AXIS2_PLACEMENT_3D ( 'NONE', #106015, #75899, #86355 ) ;
#59065=ORIENTED_EDGE ( 'NONE', *, *, #26286, .T. ) ;
#59066=CARTESIAN_POINT ( 'NONE',  ( -3.750000000000025757, 12.50000000000000000, -2.857883832488653741 ) ) ;
#59067=DIRECTION ( 'NONE',  ( 0.000000000000000000, 1.000000000000000000, 0.000000000000000000 ) ) ;
#59068=CARTESIAN_POINT ( 'NONE',  ( 4.349999999999936584, 2.500000000000000000, 6.148780366869520009 ) ) ;
#59069=ORIENTED_EDGE ( 'NONE', *, *, #47377, .T. ) ;
#59070=AXIS2_PLACEMENT_3D ( 'NONE', #121135, #102148, #91033 ) ;
#59071=CARTESIAN_POINT ( 'NONE',  ( 13.34999999999990017, 2.500000000000000000, 2.857883832488649301 ) ) ;
#59072=AXIS2_PLACEMENT_3D ( 'NONE', #68031, #40537, #117758 ) ;
#59073=AXIS2_PLACEMENT_3D ( 'NONE', #91016, #117883, #78638 ) ;
#59074=DIRECTION ( 'NONE',  ( 0.000000000000000000, 0.000000000000000000, 1.000000000000000000 ) ) ;
#59075=AXIS2_PLACEMENT_3D ( 'NONE', #119647, #78470, #109176 ) ;
#59076=VERTEX_POINT ( 'NONE', #107683 ) ;
#59077=AXIS2_PLACEMENT_3D ( 'NONE', #55598, #115801, #26145 ) ;
#59078=DIRECTION ( 'NONE',  ( -0.000000000000000000, -1.000000000000000000, -0.000000000000000000 ) ) ;
#59079=ORIENTED_EDGE ( 'NONE', *, *, #64332, .T. ) ;
#59080=CONICAL_SURFACE ( 'NONE', #44496, 0.09999999999999999167, 0.003490658503988666988 ) ;
#59081=CARTESIAN_POINT ( 'NONE',  ( 0.3999999999999568345, 2.500000000000000000, -5.022947341949754119 ) ) ;
#59082=ADVANCED_FACE ( 'NONE', ( #8812 ), #111360, .T. ) ;
#59083=EDGE_LOOP ( 'NONE', ( #54724, #38303, #4542, #111919 ) ) ;
#59085=DIRECTION ( 'NONE',  ( 0.000000000000000000, -0.000000000000000000, 1.000000000000000000 ) ) ;
#59086=ADVANCED_FACE ( 'NONE', ( #97214 ), #121984, .T. ) ;
#59087=ORIENTED_EDGE ( 'NONE', *, *, #81347, .F. ) ;
#59088=VERTEX_POINT ( 'NONE', #58592 ) ;
#59089=CARTESIAN_POINT ( 'NONE',  ( 6.699999999999930012, 2.500000000000000000, -4.330127018922201643 ) ) ;
#59090=DIRECTION ( 'NONE',  ( -0.000000000000000000, -1.000000000000000000, -0.000000000000000000 ) ) ;
#59091=ORIENTED_EDGE ( 'NONE', *, *, #2434, .T. ) ;
#59092=AXIS2_PLACEMENT_3D ( 'NONE', #78874, #38967, #108937 ) ;
#59094=DIRECTION ( 'NONE',  ( 0.000000000000000000, 0.000000000000000000, -1.000000000000000000 ) ) ;
#59095=CARTESIAN_POINT ( 'NONE',  ( 7.099999999999928590, 12.50000000000000000, -4.330127018922201643 ) ) ;
#59097=DIRECTION ( 'NONE',  ( -4.274815082592931898E-19, -0.9999939076577903929, -0.003490651415223739937 ) ) ;
#59098=DIRECTION ( 'NONE',  ( 0.000000000000000000, 0.000000000000000000, 1.000000000000000000 ) ) ;
#59099=CARTESIAN_POINT ( 'NONE',  ( -8.550000000000007816, 2.500000000000000000, 6.148780366869520009 ) ) ;
#59100=CONICAL_SURFACE ( 'NONE', #125881, 0.1000000000000000472, 0.003490658503988666988 ) ;
#59101=AXIS2_PLACEMENT_3D ( 'NONE', #101752, #42187, #91281 ) ;
#59102=CIRCLE ( 'NONE', #96731, 0.06509327318403745899 ) ;
#59103=ORIENTED_EDGE ( 'NONE', *, *, #2679, .T. ) ;
#59104=ORIENTED_EDGE ( 'NONE', *, *, #97906, .F. ) ;
#59106=ORIENTED_EDGE ( 'NONE', *, *, #35455, .T. ) ;
#59107=DIRECTION ( 'NONE',  ( 0.000000000000000000, -0.9999939076577903929, 0.003490651415223739937 ) ) ;
#59108=CARTESIAN_POINT ( 'NONE',  ( 0.1999999999999576006, 12.50000000000000000, -4.676537180435978769 ) ) ;
#59109=DIRECTION ( 'NONE',  ( 0.000000000000000000, 1.000000000000000000, 0.000000000000000000 ) ) ;
#59110=EDGE_LOOP ( 'NONE', ( #20128, #101882, #99228, #76282 ) ) ;
#59111=FACE_BOUND ( 'NONE', #69994, .T. ) ;
#59112=ORIENTED_EDGE ( 'NONE', *, *, #1024, .F. ) ;
#59113=VECTOR ( 'NONE', #117155, 1000.000000000000000 ) ;
#59114=CARTESIAN_POINT ( 'NONE',  ( -5.400000000000020783, 2.500000000000000000, 0.7928203230275495672 ) ) ;
#59115=DIRECTION ( 'NONE',  ( 0.000000000000000000, -0.000000000000000000, 1.000000000000000000 ) ) ;
#59116=AXIS2_PLACEMENT_3D ( 'NONE', #28740, #117730, #79136 ) ;
#59117=AXIS2_PLACEMENT_3D ( 'NONE', #93096, #123199, #63631 ) ;
#59118=CARTESIAN_POINT ( 'NONE',  ( -1.250000000000035749, 2.500000000000000000, -7.288010851410854585 ) ) ;
#59119=AXIS2_PLACEMENT_3D ( 'NONE', #123264, #33602, #91874 ) ;
#59120=CARTESIAN_POINT ( 'NONE',  ( 5.649999999999934630, 2.500000000000000000, 6.148780366869520897 ) ) ;
#59121=FACE_OUTER_BOUND ( 'NONE', #33846, .T. ) ;
#59122=FACE_OUTER_BOUND ( 'NONE', #62210, .T. ) ;
#59123=CARTESIAN_POINT ( 'NONE',  ( -0.8500000000000386136, 2.500000000000000000, 7.288010851410849256 ) ) ;
#59124=FACE_OUTER_BOUND ( 'NONE', #33760, .T. ) ;
#59125=DIRECTION ( 'NONE',  ( 0.000000000000000000, -0.9999939076577903929, 0.003490651415223739937 ) ) ;
#59126=VECTOR ( 'NONE', #59580, 1000.000000000000000 ) ;
#59127=CARTESIAN_POINT ( 'NONE',  ( 1.899999999999951283, 2.500000000000000000, -0.3464101615137782364 ) ) ;
#59128=EDGE_CURVE ( 'NONE', #89644, #9662, #117459, .T. ) ;
#59129=ORIENTED_EDGE ( 'NONE', *, *, #96084, .F. ) ;
#59130=VERTEX_POINT ( 'NONE', #17999 ) ;
#59131=ORIENTED_EDGE ( 'NONE', *, *, #20934, .F. ) ;
#59132=VECTOR ( 'NONE', #111805, 1000.000000000000000 ) ;
#59133=ORIENTED_EDGE ( 'NONE', *, *, #62288, .T. ) ;
#59134=CIRCLE ( 'NONE', #4810, 0.1000000000000000472 ) ;
#59135=CIRCLE ( 'NONE', #73681, 0.06509327318403745899 ) ;
#59136=PLANE ( 'NONE',  #3720 ) ;
#59137=FACE_OUTER_BOUND ( 'NONE', #59943, .T. ) ;
#59139=EDGE_LOOP ( 'NONE', ( #95270, #8850 ) ) ;
#59140=ORIENTED_EDGE ( 'NONE', *, *, #77750, .F. ) ;
#59141=AXIS2_PLACEMENT_3D ( 'NONE', #76481, #115741, #46355 ) ;
#59142=DIRECTION ( 'NONE',  ( 0.000000000000000000, -0.000000000000000000, 1.000000000000000000 ) ) ;
#59143=ADVANCED_FACE ( 'NONE', ( #101568 ), #86745, .T. ) ;
#59144=CARTESIAN_POINT ( 'NONE',  ( -10.65000000000000391, 12.50000000000000000, -2.511473670974873951 ) ) ;
#59145=CONICAL_SURFACE ( 'NONE', #75837, 0.1000000000000000472, 0.003490658503988666988 ) ;
#59146=LINE ( 'NONE', #119992, #18312 ) ;
#59147=CARTESIAN_POINT ( 'NONE',  ( 6.249999999999930722, 2.500000000000000000, -1.472243186433550122 ) ) ;
#59149=DIRECTION ( 'NONE',  ( -4.274815082592931898E-19, -0.9999939076577903929, -0.003490651415223739937 ) ) ;
#59150=ADVANCED_FACE ( 'NONE', ( #76935 ), #47475, .T. ) ;
#59151=FACE_OUTER_BOUND ( 'NONE', #49133, .T. ) ;
#59152=EDGE_CURVE ( 'NONE', #110699, #73698, #84410, .T. ) ;
#59154=DIRECTION ( 'NONE',  ( 0.000000000000000000, 0.000000000000000000, -1.000000000000000000 ) ) ;
#59155=ORIENTED_EDGE ( 'NONE', *, *, #68995, .F. ) ;
#59156=ORIENTED_EDGE ( 'NONE', *, *, #19104, .F. ) ;
#59157=VERTEX_POINT ( 'NONE', #37014 ) ;
#59158=PLANE ( 'NONE',  #50476 ) ;
#59159=CONICAL_SURFACE ( 'NONE', #2684, 0.1000000000000000472, 0.003490658503988666988 ) ;
#59160=VERTEX_POINT ( 'NONE', #27181 ) ;
#59161=EDGE_CURVE ( 'NONE', #70290, #10609, #57222, .T. ) ;
#59162=EDGE_LOOP ( 'NONE', ( #33522, #101944 ) ) ;
#59163=LINE ( 'NONE', #48050, #86175 ) ;
#59164=AXIS2_PLACEMENT_3D ( 'NONE', #16825, #47619, #98623 ) ;
#59165=LINE ( 'NONE', #80083, #1528 ) ;
#59166=DIRECTION ( 'NONE',  ( 0.000000000000000000, 1.000000000000000000, 0.000000000000000000 ) ) ;
#59167=AXIS2_PLACEMENT_3D ( 'NONE', #21579, #111899, #61523 ) ;
#59168=CARTESIAN_POINT ( 'NONE',  ( -6.650000000000018119, 2.500000000000000000, -7.188010851410854052 ) ) ;
#59169=CIRCLE ( 'NONE', #50839, 0.1000000000000000472 ) ;
#59170=DIRECTION ( 'NONE',  ( -0.000000000000000000, -1.000000000000000000, -0.000000000000000000 ) ) ;
#59171=ORIENTED_EDGE ( 'NONE', *, *, #68463, .F. ) ;
#59172=DIRECTION ( 'NONE',  ( 0.000000000000000000, 0.000000000000000000, -1.000000000000000000 ) ) ;
#59173=AXIS2_PLACEMENT_3D ( 'NONE', #32814, #21694, #2033 ) ;
#59174=AXIS2_PLACEMENT_3D ( 'NONE', #18126, #29263, #27960 ) ;
#59175=ORIENTED_EDGE ( 'NONE', *, *, #109533, .T. ) ;
#59176=CARTESIAN_POINT ( 'NONE',  ( -0.4000000000000392131, 2.500000000000000000, -5.022947341949754119 ) ) ;
#59177=CIRCLE ( 'NONE', #107275, 0.1000000000000002554 ) ;
#59178=VERTEX_POINT ( 'NONE', #98485 ) ;
#59180=LINE ( 'NONE', #2168, #27366 ) ;
#59181=AXIS2_PLACEMENT_3D ( 'NONE', #38551, #50280, #48341 ) ;
#59182=ORIENTED_EDGE ( 'NONE', *, *, #122033, .T. ) ;
#59183=CIRCLE ( 'NONE', #2715, 0.06509327318403745899 ) ;
#59184=FACE_OUTER_BOUND ( 'NONE', #4685, .T. ) ;
#59185=CARTESIAN_POINT ( 'NONE',  ( -2.100000000000033396, 2.500000000000000000, -3.737306695894649700 ) ) ;
#59186=ORIENTED_EDGE ( 'NONE', *, *, #52372, .T. ) ;
#59187=VECTOR ( 'NONE', #50482, 1000.000000000000000 ) ;
#59188=EDGE_CURVE ( 'NONE', #48804, #92562, #778, .T. ) ;
#59189=DIRECTION ( 'NONE',  ( 0.000000000000000000, -0.000000000000000000, 1.000000000000000000 ) ) ;
#59190=ORIENTED_EDGE ( 'NONE', *, *, #23169, .F. ) ;
#59192=DIRECTION ( 'NONE',  ( 0.000000000000000000, -0.000000000000000000, 1.000000000000000000 ) ) ;
#59193=CARTESIAN_POINT ( 'NONE',  ( -9.400000000000007461, 2.500000000000000000, 4.676537180435972552 ) ) ;
#59194=EDGE_CURVE ( 'NONE', #43418, #116689, #88010, .T. ) ;
#59195=PLANE ( 'NONE',  #10399 ) ;
#59196=PLANE ( 'NONE',  #42907 ) ;
#59197=EDGE_CURVE ( 'NONE', #60736, #20798, #105246, .T. ) ;
#59198=VECTOR ( 'NONE', #93198, 1000.000000000000000 ) ;
#59199=DIRECTION ( 'NONE',  ( -0.000000000000000000, -1.000000000000000000, -0.000000000000000000 ) ) ;
#59200=ORIENTED_EDGE ( 'NONE', *, *, #118745, .T. ) ;
#59201=CARTESIAN_POINT ( 'NONE',  ( 13.09999999999990195, 2.500000000000000000, -3.983716857408426293 ) ) ;
#59202=EDGE_CURVE ( 'NONE', #122805, #117378, #118785, .T. ) ;
#59203=EDGE_CURVE ( 'NONE', #116703, #58176, #78058, .T. ) ;
#59204=EDGE_CURVE ( 'NONE', #48991, #29616, #29138, .T. ) ;
#59205=EDGE_CURVE ( 'NONE', #125412, #84079, #9101, .T. ) ;
#59206=AXIS2_PLACEMENT_3D ( 'NONE', #102979, #44065, #101706 ) ;
#59207=ORIENTED_EDGE ( 'NONE', *, *, #123836, .F. ) ;
#59208=AXIS2_PLACEMENT_3D ( 'NONE', #15270, #64394, #85322 ) ;
#59209=CARTESIAN_POINT ( 'NONE',  ( 9.999999999999916511, 2.500000000000000000, -0.5928203230275541635 ) ) ;
#59210=DIRECTION ( 'NONE',  ( 0.000000000000000000, 1.000000000000000000, 0.000000000000000000 ) ) ;
#59211=AXIS2_PLACEMENT_3D ( 'NONE', #120871, #1732, #42991 ) ;
#59213=CARTESIAN_POINT ( 'NONE',  ( 5.649999999999932854, 2.500000000000000000, 2.611473670974873151 ) ) ;
#59214=DIRECTION ( 'NONE',  ( 0.000000000000000000, 0.000000000000000000, 1.000000000000000000 ) ) ;
#59215=CARTESIAN_POINT ( 'NONE',  ( -2.950000000000029932, 2.500000000000000000, 2.065063509461097624 ) ) ;
#59217=AXIS2_PLACEMENT_3D ( 'NONE', #40902, #104142, #110888 ) ;
#59218=CARTESIAN_POINT ( 'NONE',  ( -11.84999999999999787, 12.50000000000000000, -6.841600689897074261 ) ) ;
#59219=AXIS2_PLACEMENT_3D ( 'NONE', #75728, #46944, #105193 ) ;
#59220=ORIENTED_EDGE ( 'NONE', *, *, #66978, .T. ) ;
#59221=EDGE_CURVE ( 'NONE', #73869, #38720, #82584, .T. ) ;
#59222=CIRCLE ( 'NONE', #19480, 0.1000000000000002554 ) ;
#59223=AXIS2_PLACEMENT_3D ( 'NONE', #5412, #76099, #85268 ) ;
#59224=DIRECTION ( 'NONE',  ( -0.000000000000000000, -1.000000000000000000, -0.000000000000000000 ) ) ;
#59225=LINE ( 'NONE', #80137, #78597 ) ;
#59226=CARTESIAN_POINT ( 'NONE',  ( -7.499999999999976907, 12.50000000000000000, 4.330127018922196314 ) ) ;
#59227=CIRCLE ( 'NONE', #117664, 0.06509327318403745899 ) ;
#59228=EDGE_LOOP ( 'NONE', ( #68667, #44382, #90244, #8194 ) ) ;
#59229=CARTESIAN_POINT ( 'NONE',  ( -3.350000000000031619, 12.50000000000000000, -7.253104124594891289 ) ) ;
#59230=ORIENTED_EDGE ( 'NONE', *, *, #5389, .F. ) ;
#59231=AXIS2_PLACEMENT_3D ( 'NONE', #110275, #100456, #19970 ) ;
#59232=CONICAL_SURFACE ( 'NONE', #109384, 0.1000000000000002554, 0.003490658503988666988 ) ;
#59233=ORIENTED_EDGE ( 'NONE', *, *, #6028, .T. ) ;
#59234=AXIS2_PLACEMENT_3D ( 'NONE', #39831, #30002, #127548 ) ;
#59235=CARTESIAN_POINT ( 'NONE',  ( -8.750000000000010658, 12.50000000000000000, -1.537336459617587581 ) ) ;
#59236=AXIS2_PLACEMENT_3D ( 'NONE', #65184, #95956, #45579 ) ;
#59237=EDGE_LOOP ( 'NONE', ( #31358, #81980 ) ) ;
#59238=CARTESIAN_POINT ( 'NONE',  ( 14.39999999999989555, 12.50000000000000000, 0.3464101615137736845 ) ) ;
#59239=DIRECTION ( 'NONE',  ( 0.000000000000000000, 1.000000000000000000, 0.000000000000000000 ) ) ;
#59240=ORIENTED_EDGE ( 'NONE', *, *, #76878, .F. ) ;
#59241=CARTESIAN_POINT ( 'NONE',  ( -11.05000000000000071, 12.50000000000000000, -6.906693963081112386 ) ) ;
#59242=VECTOR ( 'NONE', #45601, 1000.000000000000000 ) ;
#59243=CARTESIAN_POINT ( 'NONE',  ( -4.600000000000024514, 2.500000000000000000, 0.7928203230275495672 ) ) ;
#59244=ORIENTED_EDGE ( 'NONE', *, *, #5950, .T. ) ;
#59245=DIRECTION ( 'NONE',  ( 0.000000000000000000, 1.000000000000000000, 0.000000000000000000 ) ) ;
#59246=DIRECTION ( 'NONE',  ( 0.000000000000000000, 0.000000000000000000, 1.000000000000000000 ) ) ;
#59247=ORIENTED_EDGE ( 'NONE', *, *, #29899, .F. ) ;
#59248=EDGE_CURVE ( 'NONE', #123049, #106610, #51830, .T. ) ;
#59249=ORIENTED_EDGE ( 'NONE', *, *, #44817, .T. ) ;
#59250=VERTEX_POINT ( 'NONE', #81913 ) ;
#59251=FACE_OUTER_BOUND ( 'NONE', #74809, .T. ) ;
#59252=DIRECTION ( 'NONE',  ( 0.000000000000000000, 0.000000000000000000, 1.000000000000000000 ) ) ;
#59253=AXIS2_PLACEMENT_3D ( 'NONE', #59506, #108573, #79128 ) ;
#59254=LINE ( 'NONE', #39623, #75561 ) ;
#59255=FACE_BOUND ( 'NONE', #52169, .T. ) ;
#59256=ORIENTED_EDGE ( 'NONE', *, *, #9374, .F. ) ;
#59257=CARTESIAN_POINT ( 'NONE',  ( -6.850000000000017408, 2.500000000000000000, -2.511473670974877948 ) ) ;
#59258=DIRECTION ( 'NONE',  ( -4.274815082592931898E-19, -0.9999939076577903929, -0.003490651415223739937 ) ) ;
#59259=ORIENTED_EDGE ( 'NONE', *, *, #47338, .T. ) ;
#59260=ADVANCED_FACE ( 'NONE', ( #53117 ), #21724, .T. ) ;
#59261=DIRECTION ( 'NONE',  ( 0.000000000000000000, 0.000000000000000000, 1.000000000000000000 ) ) ;
#59262=AXIS2_PLACEMENT_3D ( 'NONE', #103153, #122798, #105735 ) ;
#59263=DIRECTION ( 'NONE',  ( 0.000000000000000000, 1.000000000000000000, 0.000000000000000000 ) ) ;
#59264=AXIS2_PLACEMENT_3D ( 'NONE', #58777, #88874, #128837 ) ;
#59265=LINE ( 'NONE', #30452, #25586 ) ;
#59266=AXIS2_PLACEMENT_3D ( 'NONE', #83339, #123252, #95729 ) ;
#59267=DIRECTION ( 'NONE',  ( 0.000000000000000000, 0.000000000000000000, 1.000000000000000000 ) ) ;
#59268=LINE ( 'NONE', #79535, #21536 ) ;
#59269=FACE_OUTER_BOUND ( 'NONE', #43522, .T. ) ;
#59271=AXIS2_PLACEMENT_3D ( 'NONE', #15046, #5886, #85106 ) ;
#59272=CIRCLE ( 'NONE', #6994, 0.06509327318403745899 ) ;
#59273=AXIS2_PLACEMENT_3D ( 'NONE', #101747, #72295, #23832 ) ;
#59274=VERTEX_POINT ( 'NONE', #74039 ) ;
#59275=VERTEX_POINT ( 'NONE', #123143 ) ;
#59276=ORIENTED_EDGE ( 'NONE', *, *, #38790, .F. ) ;
#59277=EDGE_LOOP ( 'NONE', ( #88909, #65225 ) ) ;
#59278=AXIS2_PLACEMENT_3D ( 'NONE', #64601, #5664, #25302 ) ;
#59279=ORIENTED_EDGE ( 'NONE', *, *, #81147, .T. ) ;
#59280=DIRECTION ( 'NONE',  ( -0.000000000000000000, -1.000000000000000000, -0.000000000000000000 ) ) ;
#59281=VECTOR ( 'NONE', #100838, 1000.000000000000000 ) ;
#59282=FACE_OUTER_BOUND ( 'NONE', #75821, .T. ) ;
#59283=ORIENTED_EDGE ( 'NONE', *, *, #127594, .F. ) ;
#59284=FACE_BOUND ( 'NONE', #8405, .T. ) ;
#59285=AXIS2_PLACEMENT_3D ( 'NONE', #123711, #93635, #113924 ) ;
#59286=CARTESIAN_POINT ( 'NONE',  ( -11.64999999999999680, 2.500000000000000000, 5.902370205355745192 ) ) ;
#59287=CARTESIAN_POINT ( 'NONE',  ( -4.600000000000024514, 2.500000000000000000, -0.6928203230275542523 ) ) ;
#59288=FACE_OUTER_BOUND ( 'NONE', #119174, .T. ) ;
#59289=CARTESIAN_POINT ( 'NONE',  ( -6.250000000000017764, 12.50000000000000000, 2.792790559304612064 ) ) ;
#59290=CARTESIAN_POINT ( 'NONE',  ( 3.749999999999978684, 2.500000000000000000, -2.265063509461101798 ) ) ;
#59291=CARTESIAN_POINT ( 'NONE',  ( -4.550000000000022915, 2.500000000000000000, 2.165063509461097713 ) ) ;
#59292=EDGE_LOOP ( 'NONE', ( #31219, #8249, #128486, #54327 ) ) ;
#59293=CIRCLE ( 'NONE', #94865, 0.06509327318403745899 ) ;
#59294=ORIENTED_EDGE ( 'NONE', *, *, #77516, .F. ) ;
#59295=ADVANCED_FACE ( 'NONE', ( #4622 ), #71912, .T. ) ;
#59296=VERTEX_POINT ( 'NONE', #121840 ) ;
#59297=ORIENTED_EDGE ( 'NONE', *, *, #11507, .T. ) ;
#59298=CARTESIAN_POINT ( 'NONE',  ( 2.500000000000002220, 2.500000000000000000, 9.000000000000003553 ) ) ;
#59299=DIRECTION ( 'NONE',  ( 0.000000000000000000, 0.000000000000000000, -1.000000000000000000 ) ) ;
#59300=ORIENTED_EDGE ( 'NONE', *, *, #5669, .T. ) ;
#59301=DIRECTION ( 'NONE',  ( 0.000000000000000000, 0.000000000000000000, -1.000000000000000000 ) ) ;
#59302=VECTOR ( 'NONE', #73213, 1000.000000000000000 ) ;
#59303=AXIS2_PLACEMENT_3D ( 'NONE', #85803, #24318, #83871 ) ;
#59304=EDGE_CURVE ( 'NONE', #82327, #76656, #42672, .T. ) ;
#59305=VECTOR ( 'NONE', #61653, 1000.000000000000000 ) ;
#59306=DIRECTION ( 'NONE',  ( 0.000000000000000000, 1.000000000000000000, 0.000000000000000000 ) ) ;
#59307=CARTESIAN_POINT ( 'NONE',  ( 4.149999999999939959, 2.500000000000000000, 1.572243186433545548 ) ) ;
#59309=DIRECTION ( 'NONE',  ( -0.000000000000000000, 1.000000000000000000, -0.000000000000000000 ) ) ;
#59310=FACE_OUTER_BOUND ( 'NONE', #103593, .T. ) ;
#59311=EDGE_CURVE ( 'NONE', #34432, #17665, #124221, .T. ) ;
#59312=ADVANCED_FACE ( 'NONE', ( #113314 ), #112033, .T. ) ;
#59313=FACE_OUTER_BOUND ( 'NONE', #76718, .T. ) ;
#59314=CONICAL_SURFACE ( 'NONE', #76005, 0.1000000000000000472, 0.003490658503988666988 ) ;
#59316=ORIENTED_EDGE ( 'NONE', *, *, #106575, .T. ) ;
#59317=FACE_OUTER_BOUND ( 'NONE', #52671, .T. ) ;
#59318=AXIS2_PLACEMENT_3D ( 'NONE', #97317, #89427, #119522 ) ;
#59319=CIRCLE ( 'NONE', #57136, 0.06509327318403745899 ) ;
#59320=VERTEX_POINT ( 'NONE', #43945 ) ;
#59321=AXIS2_PLACEMENT_3D ( 'NONE', #112010, #32177, #102187 ) ;
#59322=ORIENTED_EDGE ( 'NONE', *, *, #121287, .T. ) ;
#59323=DIRECTION ( 'NONE',  ( -0.000000000000000000, -1.000000000000000000, -0.000000000000000000 ) ) ;
#59324=EDGE_CURVE ( 'NONE', #100266, #119869, #7125, .T. ) ;
#59325=CARTESIAN_POINT ( 'NONE',  ( -5.400000000000023448, 12.50000000000000000, -5.022947341949754119 ) ) ;
#59326=DIRECTION ( 'NONE',  ( -0.000000000000000000, -1.000000000000000000, -0.000000000000000000 ) ) ;
#59327=EDGE_CURVE ( 'NONE', #21956, #46048, #5076, .T. ) ;
#59328=AXIS2_PLACEMENT_3D ( 'NONE', #16101, #45604, #56040 ) ;
#59329=ORIENTED_EDGE ( 'NONE', *, *, #19104, .T. ) ;
#59330=VERTEX_POINT ( 'NONE', #44581 ) ;
#59331=CARTESIAN_POINT ( 'NONE',  ( -1.700000000000035261, 12.50000000000000000, 4.395220292106234439 ) ) ;
#59332=DIRECTION ( 'NONE',  ( 0.000000000000000000, 0.000000000000000000, -1.000000000000000000 ) ) ;
#59333=AXIS2_PLACEMENT_3D ( 'NONE', #78725, #30271, #79362 ) ;
#59334=AXIS2_PLACEMENT_3D ( 'NONE', #16121, #56057, #126093 ) ;
#59335=CARTESIAN_POINT ( 'NONE',  ( 4.799999999999935874, 12.50000000000000000, 3.983716857408420964 ) ) ;
#59336=ORIENTED_EDGE ( 'NONE', *, *, #7593, .F. ) ;
#59337=DIRECTION ( 'NONE',  ( 0.000000000000000000, 0.000000000000000000, -1.000000000000000000 ) ) ;
#59338=CIRCLE ( 'NONE', #44649, 0.09999999999999982514 ) ;
#59339=VERTEX_POINT ( 'NONE', #83845 ) ;
#59340=CARTESIAN_POINT ( 'NONE',  ( 12.49999999999990585, 12.50000000000000000, -5.088040615133791356 ) ) ;
#59341=EDGE_LOOP ( 'NONE', ( #58277, #20826 ) ) ;
#59342=FACE_OUTER_BOUND ( 'NONE', #57207, .T. ) ;
#59343=DIRECTION ( 'NONE',  ( -0.000000000000000000, 1.000000000000000000, -0.000000000000000000 ) ) ;
#59344=DIRECTION ( 'NONE',  ( 0.000000000000000000, 0.000000000000000000, -1.000000000000000000 ) ) ;
#59345=DIRECTION ( 'NONE',  ( 0.000000000000000000, 1.000000000000000000, 0.000000000000000000 ) ) ;
#59346=VERTEX_POINT ( 'NONE', #52454 ) ;
#59347=CARTESIAN_POINT ( 'NONE',  ( 17.50000000000000000, -2.499999999999997335, 4.040567763474973262 ) ) ;
#59348=ORIENTED_EDGE ( 'NONE', *, *, #2514, .F. ) ;
#59349=VERTEX_POINT ( 'NONE', #92378 ) ;
#59350=AXIS2_PLACEMENT_3D ( 'NONE', #122273, #104552, #116287 ) ;
#59351=AXIS2_PLACEMENT_3D ( 'NONE', #80528, #30791, #70693 ) ;
#59352=CARTESIAN_POINT ( 'NONE',  ( -8.350000000000012079, 2.500000000000000000, -1.572243186433550211 ) ) ;
#59353=DIRECTION ( 'NONE',  ( -0.000000000000000000, 1.000000000000000000, -0.000000000000000000 ) ) ;
#59354=DIRECTION ( 'NONE',  ( -4.274815082592931898E-19, -0.9999939076577903929, -0.003490651415223739937 ) ) ;
#59355=DIRECTION ( 'NONE',  ( 0.000000000000000000, 0.000000000000000000, -1.000000000000000000 ) ) ;
#59356=FACE_OUTER_BOUND ( 'NONE', #88141, .T. ) ;
#59357=CARTESIAN_POINT ( 'NONE',  ( 0.6499999999999561684, 12.50000000000000000, 2.511473670974873507 ) ) ;
#59358=CIRCLE ( 'NONE', #13255, 0.1000000000000002554 ) ;
#59359=DIRECTION ( 'NONE',  ( -0.000000000000000000, 1.000000000000000000, -0.000000000000000000 ) ) ;
#59360=CIRCLE ( 'NONE', #63546, 0.06509327318403741736 ) ;
#59361=CARTESIAN_POINT ( 'NONE',  ( 11.64999999999990266, 2.500000000000000000, 2.165063509461097713 ) ) ;
#59362=CARTESIAN_POINT ( 'NONE',  ( -13.34999999999999076, 2.500000000000000000, -1.372243186433547812 ) ) ;
#59363=AXIS2_PLACEMENT_3D ( 'NONE', #100500, #82162, #53352 ) ;
#59364=AXIS2_PLACEMENT_3D ( 'NONE', #99598, #9915, #111993 ) ;
#59365=EDGE_CURVE ( 'NONE', #7794, #38720, #80312, .T. ) ;
#59366=EDGE_CURVE ( 'NONE', #2388, #75669, #42669, .T. ) ;
#59367=EDGE_CURVE ( 'NONE', #127628, #55240, #74042, .T. ) ;
#59368=ADVANCED_FACE ( 'NONE', ( #64212 ), #11348, .T. ) ;
#59369=CIRCLE ( 'NONE', #82346, 0.06509327318403745899 ) ;
#59370=CIRCLE ( 'NONE', #126238, 0.06509327318403745899 ) ;
#59371=CONICAL_SURFACE ( 'NONE', #117812, 0.1000000000000002554, 0.003490658503988666988 ) ;
#59372=VERTEX_POINT ( 'NONE', #74684 ) ;
#59373=ADVANCED_FACE ( 'NONE', ( #114593 ), #113764, .T. ) ;
#59374=DIRECTION ( 'NONE',  ( -0.000000000000000000, -1.000000000000000000, -0.000000000000000000 ) ) ;
#59375=CIRCLE ( 'NONE', #36381, 0.06509327318403745899 ) ;
#59376=DIRECTION ( 'NONE',  ( 0.000000000000000000, 1.000000000000000000, 0.000000000000000000 ) ) ;
#59378=DIRECTION ( 'NONE',  ( -0.000000000000000000, 1.000000000000000000, -0.000000000000000000 ) ) ;
#59379=DIRECTION ( 'NONE',  ( 0.000000000000000000, 0.000000000000000000, 1.000000000000000000 ) ) ;
#59380=VERTEX_POINT ( 'NONE', #55039 ) ;
#59381=EDGE_CURVE ( 'NONE', #47889, #62993, #104759, .T. ) ;
#59382=CARTESIAN_POINT ( 'NONE',  ( 1.449999999999951328, 2.500000000000000000, -1.818653347947326138 ) ) ;
#59383=EDGE_CURVE ( 'NONE', #121302, #108298, #92837, .T. ) ;
#59384=DIRECTION ( 'NONE',  ( -0.000000000000000000, -1.000000000000000000, -0.000000000000000000 ) ) ;
#59385=LINE ( 'NONE', #27963, #86009 ) ;
#59386=ORIENTED_EDGE ( 'NONE', *, *, #20970, .T. ) ;
#59387=( BOUNDED_SURFACE ( )  B_SPLINE_SURFACE ( 3, 2, ( 
 ( #31075, #3994, #74682 ),
 ( #60538, #114591, #30431 ),
 ( #61157, #93677, #43306 ),
 ( #64209, #103503, #34122 ) ),
 .UNSPECIFIED., .F., .F., .F. ) 
 B_SPLINE_SURFACE_WITH_KNOTS ( ( 4, 4 ),
 ( 3, 3 ),
 ( 0.000000000000000000, 0.002140783231465592188 ),
 ( 0.000000000000000000, 1.000000000000000000 ),
 .UNSPECIFIED. ) 
 GEOMETRIC_REPRESENTATION_ITEM ( )  RATIONAL_B_SPLINE_SURFACE ( (
 ( 1.000000000000000000, 0.7071067811865473507, 1.000000000000000000),
 ( 1.000000000000000000, 0.7083221553718342944, 1.000000000000000000),
 ( 1.000000000000000000, 0.7095583407460057668, 1.000000000000000000),
 ( 1.000000000000000000, 0.7108129114090289136, 1.000000000000000000) ) ) 
 REPRESENTATION_ITEM ( '' )  SURFACE ( )  );
#59388=ADVANCED_FACE ( 'NONE', ( #126362 ), #84508, .T. ) ;
#59389=AXIS2_PLACEMENT_3D ( 'NONE', #127012, #6536, #57627 ) ;
#59390=VERTEX_POINT ( 'NONE', #26871 ) ;
#59391=CARTESIAN_POINT ( 'NONE',  ( -1.250000000000001554, 12.50000000000000000, 6.495190528383297135 ) ) ;
#59392=EDGE_LOOP ( 'NONE', ( #100442, #69210, #93766, #112249 ) ) ;
#59393=EDGE_LOOP ( 'NONE', ( #109278, #63091 ) ) ;
#59394=EDGE_LOOP ( 'NONE', ( #41365, #11183 ) ) ;
#59395=DIRECTION ( 'NONE',  ( 0.000000000000000000, 0.000000000000000000, 1.000000000000000000 ) ) ;
#59396=FACE_OUTER_BOUND ( 'NONE', #120366, .T. ) ;
#59397=DIRECTION ( 'NONE',  ( -4.274815082592931898E-19, -0.9999939076577903929, -0.003490651415223739937 ) ) ;
#59398=DIRECTION ( 'NONE',  ( -0.000000000000000000, -1.000000000000000000, -0.000000000000000000 ) ) ;
#59399=AXIS2_PLACEMENT_3D ( 'NONE', #60225, #39306, #88346 ) ;
#59400=VERTEX_POINT ( 'NONE', #66780 ) ;
#59401=DIRECTION ( 'NONE',  ( 0.000000000000000000, 1.000000000000000000, 0.000000000000000000 ) ) ;
#59402=EDGE_LOOP ( 'NONE', ( #122708, #67360 ) ) ;
#59403=CARTESIAN_POINT ( 'NONE',  ( 11.89999999999990798, 2.500000000000000000, -3.983716857408426293 ) ) ;
#59404=DIRECTION ( 'NONE',  ( 0.000000000000000000, 0.000000000000000000, 1.000000000000000000 ) ) ;
#59405=DIRECTION ( 'NONE',  ( 0.000000000000000000, -0.9999939076577903929, 0.003490651415223739937 ) ) ;
#59407=CIRCLE ( 'NONE', #15450, 0.09999999999999999167 ) ;
#59408=VERTEX_POINT ( 'NONE', #86423 ) ;
#59409=CIRCLE ( 'NONE', #2958, 0.06509327318403741736 ) ;
#59410=ORIENTED_EDGE ( 'NONE', *, *, #634, .T. ) ;
#59411=ORIENTED_EDGE ( 'NONE', *, *, #7037, .T. ) ;
#59412=ORIENTED_EDGE ( 'NONE', *, *, #40306, .T. ) ;
#59413=EDGE_LOOP ( 'NONE', ( #102799, #20381 ) ) ;
#59414=CARTESIAN_POINT ( 'NONE',  ( 4.799999999999937650, 12.50000000000000000, -0.3464101615137782364 ) ) ;
#59415=DIRECTION ( 'NONE',  ( 0.000000000000000000, 0.000000000000000000, -1.000000000000000000 ) ) ;
#59416=DIRECTION ( 'NONE',  ( 0.000000000000000000, -0.000000000000000000, 1.000000000000000000 ) ) ;
#59417=FACE_BOUND ( 'NONE', #115439, .T. ) ;
#59418=CARTESIAN_POINT ( 'NONE',  ( -9.800000000000007816, 12.50000000000000000, -3.983716857408421852 ) ) ;
#59419=CARTESIAN_POINT ( 'NONE',  ( 5.599999999999933031, 12.50000000000000000, 0.4115034346978109769 ) ) ;
#59420=DIRECTION ( 'NONE',  ( 0.000000000000000000, 0.000000000000000000, 1.000000000000000000 ) ) ;
#59421=CARTESIAN_POINT ( 'NONE',  ( -1.900000000000034994, 2.500000000000000000, -0.3464101615137783474 ) ) ;
#59422=EDGE_CURVE ( 'NONE', #22780, #29957, #103298, .T. ) ;
#59423=CONICAL_SURFACE ( 'NONE', #23902, 0.09999999999999982514, 0.003490658503988666988 ) ;
#59425=CIRCLE ( 'NONE', #74061, 0.09999999999999982514 ) ;
#59426=DIRECTION ( 'NONE',  ( 0.000000000000000000, 1.000000000000000000, 0.000000000000000000 ) ) ;
#59428=AXIS2_PLACEMENT_3D ( 'NONE', #7404, #39490, #98364 ) ;
#59429=DIRECTION ( 'NONE',  ( 0.000000000000000000, 0.000000000000000000, -1.000000000000000000 ) ) ;
#59430=CIRCLE ( 'NONE', #40653, 0.1000000000000002554 ) ;
#59431=DIRECTION ( 'NONE',  ( 0.000000000000000000, 0.000000000000000000, -1.000000000000000000 ) ) ;
#59432=ORIENTED_EDGE ( 'NONE', *, *, #126252, .T. ) ;
#59433=ORIENTED_EDGE ( 'NONE', *, *, #47155, .F. ) ;
#59434=VERTEX_POINT ( 'NONE', #87711 ) ;
#59435=ORIENTED_EDGE ( 'NONE', *, *, #105991, .F. ) ;
#59436=DIRECTION ( 'NONE',  ( 0.000000000000000000, 0.000000000000000000, 1.000000000000000000 ) ) ;
#59437=DIRECTION ( 'NONE',  ( 0.000000000000000000, 1.000000000000000000, 0.000000000000000000 ) ) ;
#59438=FACE_BOUND ( 'NONE', #127993, .T. ) ;
#59439=CARTESIAN_POINT ( 'NONE',  ( -3.100000000000028511, 12.50000000000000000, -3.983716857408426293 ) ) ;
#59440=CIRCLE ( 'NONE', #44852, 0.06509327318403745899 ) ;
#59441=AXIS2_PLACEMENT_3D ( 'NONE', #95379, #105837, #67168 ) ;
#59442=VERTEX_POINT ( 'NONE', #17005 ) ;
#59443=FACE_OUTER_BOUND ( 'NONE', #99516, .T. ) ;
#59444=CIRCLE ( 'NONE', #15489, 0.06509327318403745899 ) ;
#59445=PLANE ( 'NONE',  #28628 ) ;
#59446=DIRECTION ( 'NONE',  ( 0.000000000000000000, 0.000000000000000000, 1.000000000000000000 ) ) ;
#59447=DIRECTION ( 'NONE',  ( -0.000000000000000000, 1.000000000000000000, -0.000000000000000000 ) ) ;
#59448=ORIENTED_EDGE ( 'NONE', *, *, #65791, .F. ) ;
#59449=DIRECTION ( 'NONE',  ( -0.000000000000000000, -1.000000000000000000, -0.000000000000000000 ) ) ;
#59450=VECTOR ( 'NONE', #108148, 1000.000000000000000 ) ;
#59451=AXIS2_PLACEMENT_3D ( 'NONE', #69140, #10850, #9595 ) ;
#59452=VECTOR ( 'NONE', #51445, 1000.000000000000000 ) ;
#59453=AXIS2_PLACEMENT_3D ( 'NONE', #9242, #89729, #60911 ) ;
#59454=ORIENTED_EDGE ( 'NONE', *, *, #104769, .T. ) ;
#59455=ORIENTED_EDGE ( 'NONE', *, *, #10115, .F. ) ;
#59456=DIRECTION ( 'NONE',  ( 0.000000000000000000, 0.000000000000000000, -1.000000000000000000 ) ) ;
#59457=CARTESIAN_POINT ( 'NONE',  ( 9.199999999999919353, 2.500000000000000000, -2.276824562219559311E-15 ) ) ;
#59459=CIRCLE ( 'NONE', #25694, 0.1000000000000002554 ) ;
#59460=AXIS2_PLACEMENT_3D ( 'NONE', #27428, #107935, #17613 ) ;
#59461=VECTOR ( 'NONE', #107386, 1000.000000000000000 ) ;
#59462=EDGE_CURVE ( 'NONE', #115836, #105649, #86556, .T. ) ;
#59463=CARTESIAN_POINT ( 'NONE',  ( 2.499999999999983569, 2.500000000000000000, -4.330127018922201643 ) ) ;
#59464=DIRECTION ( 'NONE',  ( 0.000000000000000000, 0.000000000000000000, -1.000000000000000000 ) ) ;
#59465=VERTEX_POINT ( 'NONE', #36054 ) ;
#59466=CARTESIAN_POINT ( 'NONE',  ( 9.349999999999916156, 12.50000000000000000, -1.753560074763288679 ) ) ;
#59467=AXIS2_PLACEMENT_3D ( 'NONE', #31979, #129549, #9748 ) ;
#59468=ORIENTED_EDGE ( 'NONE', *, *, #2589, .T. ) ;
#59469=EDGE_CURVE ( 'NONE', #97052, #6303, #884, .T. ) ;
#59470=PLANE ( 'NONE',  #57911 ) ;
#59471=ADVANCED_FACE ( 'NONE', ( #15745 ), #126278, .T. ) ;
#59472=EDGE_LOOP ( 'NONE', ( #69974, #63110 ) ) ;
#59473=DIRECTION ( 'NONE',  ( 0.000000000000000000, 0.000000000000000000, 1.000000000000000000 ) ) ;
#59474=FACE_BOUND ( 'NONE', #45580, .T. ) ;
#59475=ORIENTED_EDGE ( 'NONE', *, *, #51530, .T. ) ;
#59476=CARTESIAN_POINT ( 'NONE',  ( 6.699999999999930012, 2.500000000000000000, 4.430127018922196847 ) ) ;
#59477=ORIENTED_EDGE ( 'NONE', *, *, #40414, .F. ) ;
#59478=FACE_OUTER_BOUND ( 'NONE', #90374, .T. ) ;
#59480=EDGE_CURVE ( 'NONE', #108547, #26951, #96891, .T. ) ;
#59481=ADVANCED_FACE ( 'NONE', ( #77890 ), #46861, .T. ) ;
#59482=DIRECTION ( 'NONE',  ( -0.000000000000000000, -1.000000000000000000, -0.000000000000000000 ) ) ;
#59483=EDGE_CURVE ( 'NONE', #35498, #109299, #55681, .T. ) ;
#59484=CARTESIAN_POINT ( 'NONE',  ( -5.200000000000022382, 12.50000000000000000, 0.4115034346978109769 ) ) ;
#59485=ADVANCED_FACE ( 'NONE', ( #7863 ), #17593, .T. ) ;
#59486=EDGE_CURVE ( 'NONE', #5786, #12706, #96239, .T. ) ;
#59487=LINE ( 'NONE', #39195, #3527 ) ;
#59488=VECTOR ( 'NONE', #15852, 1000.000000000000000 ) ;
#59489=EDGE_LOOP ( 'NONE', ( #18277, #57732, #92641, #4978 ) ) ;
#59490=VERTEX_POINT ( 'NONE', #67406 ) ;
#59491=ORIENTED_EDGE ( 'NONE', *, *, #98930, .T. ) ;
#59492=DIRECTION ( 'NONE',  ( -0.000000000000000000, 1.000000000000000000, -0.000000000000000000 ) ) ;
#59493=PLANE ( 'NONE',  #5546 ) ;
#59494=DIRECTION ( 'NONE',  ( -4.274815082592931898E-19, -0.9999939076577903929, -0.003490651415223739937 ) ) ;
#59495=ORIENTED_EDGE ( 'NONE', *, *, #13017, .F. ) ;
#59496=VERTEX_POINT ( 'NONE', #115889 ) ;
#59497=ORIENTED_EDGE ( 'NONE', *, *, #107139, .T. ) ;
#59498=EDGE_CURVE ( 'NONE', #70678, #76293, #61532, .T. ) ;
#59499=CARTESIAN_POINT ( 'NONE',  ( -4.150000000000024336, 2.500000000000000000, -2.957883832488653830 ) ) ;
#59500=AXIS2_PLACEMENT_3D ( 'NONE', #105788, #26588, #65855 ) ;
#59501=DIRECTION ( 'NONE',  ( -0.000000000000000000, 1.000000000000000000, -0.000000000000000000 ) ) ;
#59503=FACE_OUTER_BOUND ( 'NONE', #83171, .T. ) ;
#59504=CARTESIAN_POINT ( 'NONE',  ( 8.749999999999920064, 12.50000000000000000, -2.857883832488653741 ) ) ;
#59505=CARTESIAN_POINT ( 'NONE',  ( -10.60000000000000320, 12.50000000000000000, -3.983716857408421852 ) ) ;
#59506=CARTESIAN_POINT ( 'NONE',  ( 0.5999999999999555689, 12.50000000000000000, 4.676537180435972552 ) ) ;
#59507=CARTESIAN_POINT ( 'NONE',  ( -12.89999999999999147, 12.50000000000000000, 1.843143693225357538E-15 ) ) ;
#59508=ORIENTED_EDGE ( 'NONE', *, *, #72228, .T. ) ;
#59509=ORIENTED_EDGE ( 'NONE', *, *, #110417, .T. ) ;
#59510=AXIS2_PLACEMENT_3D ( 'NONE', #103653, #23801, #22530 ) ;
#59511=DIRECTION ( 'NONE',  ( 0.000000000000000000, 1.000000000000000000, 0.000000000000000000 ) ) ;
#59512=AXIS2_PLACEMENT_3D ( 'NONE', #64868, #113989, #17027 ) ;
#59513=DIRECTION ( 'NONE',  ( -0.000000000000000000, -1.000000000000000000, -0.000000000000000000 ) ) ;
#59514=ORIENTED_EDGE ( 'NONE', *, *, #17923, .T. ) ;
#59515=ORIENTED_EDGE ( 'NONE', *, *, #73148, .T. ) ;
#59517=DIRECTION ( 'NONE',  ( 0.000000000000000000, 0.000000000000000000, -1.000000000000000000 ) ) ;
#59518=DIRECTION ( 'NONE',  ( 0.000000000000000000, 0.000000000000000000, -1.000000000000000000 ) ) ;
#59519=DIRECTION ( 'NONE',  ( -0.000000000000000000, -1.000000000000000000, -0.000000000000000000 ) ) ;
#59520=CIRCLE ( 'NONE', #7232, 0.1000000000000000472 ) ;
#59521=CARTESIAN_POINT ( 'NONE',  ( 4.399999999999939071, 2.500000000000000000, -0.3464101615137782364 ) ) ;
#59522=CONICAL_SURFACE ( 'NONE', #53242, 0.1000000000000000056, 0.003490658503988666988 ) ;
#59523=PLANE ( 'NONE',  #122152 ) ;
#59524=DIRECTION ( 'NONE',  ( 0.000000000000000000, 0.000000000000000000, -1.000000000000000000 ) ) ;
#59525=AXIS2_PLACEMENT_3D ( 'NONE', #125108, #5958, #34158 ) ;
#59526=ADVANCED_FACE ( 'NONE', ( #75318 ), #90759, .T. ) ;
#59527=ADVANCED_FACE ( 'NONE', ( #107361 ), #95614, .T. ) ;
#59528=CARTESIAN_POINT ( 'NONE',  ( -8.300000000000011369, 2.500000000000000000, -4.430127018922202176 ) ) ;
#59529=ORIENTED_EDGE ( 'NONE', *, *, #54994, .T. ) ;
#59530=EDGE_CURVE ( 'NONE', #33059, #10801, #65627, .T. ) ;
#59531=ORIENTED_EDGE ( 'NONE', *, *, #107367, .F. ) ;
#59532=VERTEX_POINT ( 'NONE', #119120 ) ;
#59533=EDGE_CURVE ( 'NONE', #21628, #82736, #69839, .T. ) ;
#59534=EDGE_LOOP ( 'NONE', ( #93122, #36432 ) ) ;
#59535=FACE_OUTER_BOUND ( 'NONE', #115308, .T. ) ;
#59536=CARTESIAN_POINT ( 'NONE',  ( -6.050000000000018474, 2.500000000000000000, 6.841600689897072485 ) ) ;
#59538=VERTEX_POINT ( 'NONE', #70026 ) ;
#59539=ADVANCED_FACE ( 'NONE', ( #1275 ), #78354, .T. ) ;
#59540=CARTESIAN_POINT ( 'NONE',  ( 7.049999999999928768, 2.500000000000000000, -2.265063509461101798 ) ) ;
#59541=DIRECTION ( 'NONE',  ( -4.274815082592931898E-19, -0.9999939076577903929, -0.003490651415223739937 ) ) ;
#59543=AXIS2_PLACEMENT_3D ( 'NONE', #56881, #87009, #65432 ) ;
#59544=CIRCLE ( 'NONE', #78398, 0.06509327318403745899 ) ;
#59546=CARTESIAN_POINT ( 'NONE',  ( 10.84999999999991260, 2.500000000000000000, 6.395190528383296602 ) ) ;
#59547=EDGE_LOOP ( 'NONE', ( #43860, #112434 ) ) ;
#59548=AXIS2_PLACEMENT_3D ( 'NONE', #48066, #119363, #67682 ) ;
#59549=AXIS2_PLACEMENT_3D ( 'NONE', #87439, #118201, #48833 ) ;
#59550=DIRECTION ( 'NONE',  ( 0.000000000000000000, 0.000000000000000000, 1.000000000000000000 ) ) ;
#59551=EDGE_CURVE ( 'NONE', #11954, #74899, #105440, .T. ) ;
#59552=DIRECTION ( 'NONE',  ( 0.000000000000000000, 0.000000000000000000, -1.000000000000000000 ) ) ;
#59553=VERTEX_POINT ( 'NONE', #48441 ) ;
#59554=CONICAL_SURFACE ( 'NONE', #72051, 0.09999999999999982514, 0.003490658503988666988 ) ;
#59555=CONICAL_SURFACE ( 'NONE', #24017, 0.09999999999999982514, 0.003490658503988666988 ) ;
#59556=AXIS2_PLACEMENT_3D ( 'NONE', #87946, #106952, #17264 ) ;
#59557=ORIENTED_EDGE ( 'NONE', *, *, #96781, .T. ) ;
#59558=ORIENTED_EDGE ( 'NONE', *, *, #28440, .T. ) ;
#59559=ORIENTED_EDGE ( 'NONE', *, *, #63851, .T. ) ;
#59561=DIRECTION ( 'NONE',  ( 0.000000000000000000, 0.000000000000000000, -1.000000000000000000 ) ) ;
#59562=CONICAL_SURFACE ( 'NONE', #80476, 0.1000000000000002554, 0.003490658503988666988 ) ;
#59563=CIRCLE ( 'NONE', #42836, 0.09999999999999982514 ) ;
#59564=VECTOR ( 'NONE', #90068, 1000.000000000000000 ) ;
#59565=ORIENTED_EDGE ( 'NONE', *, *, #98739, .T. ) ;
#59566=LINE ( 'NONE', #90926, #41221 ) ;
#59567=CARTESIAN_POINT ( 'NONE',  ( -4.150000000000027889, 12.50000000000000000, -6.495190528383302464 ) ) ;
#59568=CARTESIAN_POINT ( 'NONE',  ( -12.49999999999995737, 2.500000000000000000, 4.230127018922196669 ) ) ;
#59569=DIRECTION ( 'NONE',  ( -0.000000000000000000, -1.000000000000000000, -0.000000000000000000 ) ) ;
#59570=EDGE_CURVE ( 'NONE', #55527, #95554, #80409, .T. ) ;
#59571=EDGE_LOOP ( 'NONE', ( #58075, #75522, #4738, #41900 ) ) ;
#59572=DIRECTION ( 'NONE',  ( 0.000000000000000000, -0.9999939076577903929, 0.003490651415223739937 ) ) ;
#59573=VERTEX_POINT ( 'NONE', #81139 ) ;
#59574=EDGE_LOOP ( 'NONE', ( #32147, #115219, #106934, #27579 ) ) ;
#59575=CARTESIAN_POINT ( 'NONE',  ( -2.950000000000030376, 12.50000000000000000, 6.495190528383297135 ) ) ;
#59576=DIRECTION ( 'NONE',  ( 0.000000000000000000, 0.000000000000000000, 1.000000000000000000 ) ) ;
#59577=FACE_BOUND ( 'NONE', #85920, .T. ) ;
#59578=CARTESIAN_POINT ( 'NONE',  ( -6.505213034913026604E-15, 2.500000000000000000, 4.430127018922196847 ) ) ;
#59579=CIRCLE ( 'NONE', #45077, 0.1000000000000000472 ) ;
#59580=DIRECTION ( 'NONE',  ( 0.000000000000000000, -0.9999939076577903929, 0.003490651415223739937 ) ) ;
#59581=CARTESIAN_POINT ( 'NONE',  ( 3.299999999999942979, 12.50000000000000000, 4.265033745738159077 ) ) ;
#59582=ADVANCED_FACE ( 'NONE', ( #89662 ), #111698, .T. ) ;
#59583=VERTEX_POINT ( 'NONE', #59587 ) ;
#59584=CARTESIAN_POINT ( 'NONE',  ( -3.550000000000028244, 2.500000000000000000, -1.818653347947326138 ) ) ;
#59585=DIRECTION ( 'NONE',  ( -0.000000000000000000, -1.000000000000000000, -0.000000000000000000 ) ) ;
#59586=DIRECTION ( 'NONE',  ( 0.000000000000000000, 1.000000000000000000, 0.000000000000000000 ) ) ;
#59587=CARTESIAN_POINT ( 'NONE',  ( 6.649999999999931966, 2.500000000000000000, -7.088010851410853519 ) ) ;
#59588=ORIENTED_EDGE ( 'NONE', *, *, #113424, .T. ) ;
#59589=CIRCLE ( 'NONE', #76279, 0.06509327318403745899 ) ;
#59590=AXIS2_PLACEMENT_3D ( 'NONE', #112375, #3695, #2385 ) ;
#59591=DIRECTION ( 'NONE',  ( -0.000000000000000000, -1.000000000000000000, -0.000000000000000000 ) ) ;
#59592=DIRECTION ( 'NONE',  ( -0.000000000000000000, -1.000000000000000000, -0.000000000000000000 ) ) ;
#59593=ORIENTED_EDGE ( 'NONE', *, *, #34857, .T. ) ;
#59594=VERTEX_POINT ( 'NONE', #119759 ) ;
#59595=DIRECTION ( 'NONE',  ( 0.000000000000000000, 1.000000000000000000, 0.000000000000000000 ) ) ;
#59596=EDGE_CURVE ( 'NONE', #36965, #6322, #92926, .T. ) ;
#59597=CARTESIAN_POINT ( 'NONE',  ( -12.09999999999999609, 2.500000000000000000, -4.230127018922199333 ) ) ;
#59598=FACE_BOUND ( 'NONE', #11063, .T. ) ;
#59599=CARTESIAN_POINT ( 'NONE',  ( -14.14999999999998792, 2.500000000000000000, 2.857883832488652853 ) ) ;
#59600=AXIS2_PLACEMENT_3D ( 'NONE', #4772, #93192, #114741 ) ;
#59601=DIRECTION ( 'NONE',  ( 0.000000000000000000, -0.9999939076577903929, 0.003490651415223739937 ) ) ;
#59602=AXIS2_PLACEMENT_3D ( 'NONE', #51700, #122374, #71316 ) ;
#59604=DIRECTION ( 'NONE',  ( -0.000000000000000000, 1.000000000000000000, -0.000000000000000000 ) ) ;
#59606=ORIENTED_EDGE ( 'NONE', *, *, #46619, .F. ) ;
#59608=DIRECTION ( 'NONE',  ( 0.000000000000000000, 0.000000000000000000, 1.000000000000000000 ) ) ;
#59609=AXIS2_PLACEMENT_3D ( 'NONE', #120416, #44919, #114288 ) ;
#59610=VECTOR ( 'NONE', #21263, 1000.000000000000000 ) ;
#59611=DIRECTION ( 'NONE',  ( 0.000000000000000000, -0.000000000000000000, 1.000000000000000000 ) ) ;
#59612=CARTESIAN_POINT ( 'NONE',  ( -6.850000000000013856, 2.500000000000000000, 2.611473670974873151 ) ) ;
#59613=VERTEX_POINT ( 'NONE', #51041 ) ;
#59614=ADVANCED_FACE ( 'NONE', ( #99492 ), #26025, .T. ) ;
#59616=CARTESIAN_POINT ( 'NONE',  ( -10.85000000000000142, 12.50000000000000000, -7.122917578226813262 ) ) ;
#59617=CARTESIAN_POINT ( 'NONE',  ( -5.850000000000019185, 12.50000000000000000, 6.495190528383297135 ) ) ;
#59618=DIRECTION ( 'NONE',  ( 0.000000000000000000, 0.000000000000000000, -1.000000000000000000 ) ) ;
#59619=EDGE_LOOP ( 'NONE', ( #32213, #85282 ) ) ;
#59620=ORIENTED_EDGE ( 'NONE', *, *, #70368, .T. ) ;
#59621=PLANE ( 'NONE',  #118314 ) ;
#59622=CONICAL_SURFACE ( 'NONE', #49151, 0.09999999999999982514, 0.003490658503988666988 ) ;
#59623=ORIENTED_EDGE ( 'NONE', *, *, #25323, .T. ) ;
#59624=DIRECTION ( 'NONE',  ( 0.000000000000000000, 1.000000000000000000, 0.000000000000000000 ) ) ;
#59625=PLANE ( 'NONE',  #49497 ) ;
#59626=CIRCLE ( 'NONE', #70065, 0.1000000000000002554 ) ;
#59627=DIRECTION ( 'NONE',  ( 0.000000000000000000, 0.000000000000000000, 1.000000000000000000 ) ) ;
#59628=VERTEX_POINT ( 'NONE', #18969 ) ;
#59629=CARTESIAN_POINT ( 'NONE',  ( 13.94999999999989448, 12.50000000000000000, -2.576566944158915184 ) ) ;
#59630=DIRECTION ( 'NONE',  ( 0.000000000000000000, 0.000000000000000000, 1.000000000000000000 ) ) ;
#59632=EDGE_CURVE ( 'NONE', #45780, #31546, #15534, .T. ) ;
#59633=EDGE_CURVE ( 'NONE', #106056, #105502, #49757, .T. ) ;
#59635=CARTESIAN_POINT ( 'NONE',  ( -9.800000000000006040, 2.500000000000000000, -4.576537180435973795 ) ) ;
#59636=EDGE_CURVE ( 'NONE', #88688, #72798, #21830, .T. ) ;
#59637=EDGE_CURVE ( 'NONE', #25624, #95786, #50376, .T. ) ;
#59638=DIRECTION ( 'NONE',  ( 0.000000000000000000, -0.000000000000000000, 1.000000000000000000 ) ) ;
#59639=AXIS2_PLACEMENT_3D ( 'NONE', #91842, #128057, #1512 ) ;
#59640=ORIENTED_EDGE ( 'NONE', *, *, #75384, .T. ) ;
#59641=CIRCLE ( 'NONE', #103527, 0.06509327318403745899 ) ;
#59642=ORIENTED_EDGE ( 'NONE', *, *, #83433, .F. ) ;
#59643=AXIS2_PLACEMENT_3D ( 'NONE', #68168, #88449, #7308 ) ;
#59644=FACE_OUTER_BOUND ( 'NONE', #99707, .T. ) ;
#59645=VERTEX_POINT ( 'NONE', #121047 ) ;
#59647=AXIS2_PLACEMENT_3D ( 'NONE', #45041, #103308, #14882 ) ;
#59648=VERTEX_POINT ( 'NONE', #80501 ) ;
#59649=ORIENTED_EDGE ( 'NONE', *, *, #95607, .T. ) ;
#59650=ORIENTED_EDGE ( 'NONE', *, *, #33077, .T. ) ;
#59651=ADVANCED_FACE ( 'NONE', ( #120414 ), #36503, .T. ) ;
#59652=CARTESIAN_POINT ( 'NONE',  ( 87.49999999999998579, 1.433398978532516743, -7.395196794792771477 ) ) ;
#59653=ADVANCED_FACE ( 'NONE', ( #33341 ), #31398, .T. ) ;
#59654=AXIS2_PLACEMENT_3D ( 'NONE', #45509, #4251, #73646 ) ;
#59655=DIRECTION ( 'NONE',  ( -0.000000000000000000, 1.000000000000000000, -0.000000000000000000 ) ) ;
#59656=AXIS2_PLACEMENT_3D ( 'NONE', #125272, #8064, #95169 ) ;
#59657=EDGE_CURVE ( 'NONE', #79041, #93285, #82464, .T. ) ;
#59658=CARTESIAN_POINT ( 'NONE',  ( -0.8000000000000315747, 12.50000000000000000, 0.06509327318403743123 ) ) ;
#59659=DIRECTION ( 'NONE',  ( -0.000000000000000000, -1.000000000000000000, -0.000000000000000000 ) ) ;
#59660=CARTESIAN_POINT ( 'NONE',  ( 12.29999999999990656, 2.500000000000000000, -4.776537180435977525 ) ) ;
#59661=CARTESIAN_POINT ( 'NONE',  ( 6.049999999999935874, 12.50000000000000000, -6.906693963081115051 ) ) ;
#59662=CIRCLE ( 'NONE', #111861, 0.06509327318403745899 ) ;
#59663=DIRECTION ( 'NONE',  ( 0.000000000000000000, 0.000000000000000000, 1.000000000000000000 ) ) ;
#59664=LINE ( 'NONE', #128392, #3004 ) ;
#59665=CARTESIAN_POINT ( 'NONE',  ( -5.800000000000022027, 2.500000000000000000, -4.230127018922201998 ) ) ;
#59666=ORIENTED_EDGE ( 'NONE', *, *, #3046, .T. ) ;
#59667=EDGE_LOOP ( 'NONE', ( #64119, #49892 ) ) ;
#59668=DIRECTION ( 'NONE',  ( -0.000000000000000000, -1.000000000000000000, -0.000000000000000000 ) ) ;
#59669=ORIENTED_EDGE ( 'NONE', *, *, #97851, .F. ) ;
#59670=EDGE_LOOP ( 'NONE', ( #8367, #110890 ) ) ;
#59671=DIRECTION ( 'NONE',  ( -4.274815082592931898E-19, -0.9999939076577903929, -0.003490651415223739937 ) ) ;
#59672=CARTESIAN_POINT ( 'NONE',  ( -4.200000000000025935, 12.50000000000000000, 4.395220292106234439 ) ) ;
#59673=DIRECTION ( 'NONE',  ( -0.000000000000000000, -1.000000000000000000, -0.000000000000000000 ) ) ;
#59674=DIRECTION ( 'NONE',  ( 0.000000000000000000, 1.000000000000000000, 0.000000000000000000 ) ) ;
#59675=DIRECTION ( 'NONE',  ( 0.000000000000000000, 0.000000000000000000, 1.000000000000000000 ) ) ;
#59676=ORIENTED_EDGE ( 'NONE', *, *, #122145, .F. ) ;
#59677=AXIS2_PLACEMENT_3D ( 'NONE', #13858, #74724, #123807 ) ;
#59678=VECTOR ( 'NONE', #111565, 1000.000000000000000 ) ;
#59679=EDGE_LOOP ( 'NONE', ( #73629, #125948, #18140, #36036 ) ) ;
#59680=DIRECTION ( 'NONE',  ( 0.000000000000000000, 0.000000000000000000, 1.000000000000000000 ) ) ;
#59681=ORIENTED_EDGE ( 'NONE', *, *, #40293, .T. ) ;
#59682=CARTESIAN_POINT ( 'NONE',  ( 1.449999999999951328, 2.500000000000000000, 2.511473670974873507 ) ) ;
#59683=EDGE_LOOP ( 'NONE', ( #122723, #69065 ) ) ;
#59685=ORIENTED_EDGE ( 'NONE', *, *, #85425, .F. ) ;
#59686=DIRECTION ( 'NONE',  ( 0.000000000000000000, -0.000000000000000000, 1.000000000000000000 ) ) ;
#59687=CARTESIAN_POINT ( 'NONE',  ( -2.500000000000030642, 2.500000000000000000, -5.122947341949753763 ) ) ;
#59688=AXIS2_PLACEMENT_3D ( 'NONE', #83834, #11873, #102822 ) ;
#59689=ADVANCED_FACE ( 'NONE', ( #93526 ), #84350, .T. ) ;
#59690=CARTESIAN_POINT ( 'NONE',  ( -7.500000000000001776, 1.500000000000000000, -8.999999999999998224 ) ) ;
#59691=LINE ( 'NONE', #6653, #109211 ) ;
#59692=AXIS2_PLACEMENT_3D ( 'NONE', #16095, #64569, #44946 ) ;
#59693=ADVANCED_FACE ( 'NONE', ( #83074 ), #109645, .T. ) ;
#59694=DIRECTION ( 'NONE',  ( -4.274815082592931898E-19, -0.9999939076577903929, -0.003490651415223739937 ) ) ;
#59695=VERTEX_POINT ( 'NONE', #82438 ) ;
#59696=CARTESIAN_POINT ( 'NONE',  ( 8.549999999999922551, 12.50000000000000000, -6.148780366869526226 ) ) ;
#59697=DIRECTION ( 'NONE',  ( 0.000000000000000000, 0.000000000000000000, 1.000000000000000000 ) ) ;
#59698=DIRECTION ( 'NONE',  ( -0.000000000000000000, -1.000000000000000000, -0.000000000000000000 ) ) ;
#59699=DIRECTION ( 'NONE',  ( 0.000000000000000000, 1.000000000000000000, 0.000000000000000000 ) ) ;
#59700=ADVANCED_FACE ( 'NONE', ( #92221 ), #78264, .T. ) ;
#59701=DIRECTION ( 'NONE',  ( -4.274815082592931898E-19, -0.9999939076577903929, -0.003490651415223739937 ) ) ;
#59702=VERTEX_POINT ( 'NONE', #102688 ) ;
#59703=CONICAL_SURFACE ( 'NONE', #76404, 0.1000000000000000056, 0.003490658503988666988 ) ;
#59704=AXIS2_PLACEMENT_3D ( 'NONE', #12572, #82631, #61038 ) ;
#59705=ORIENTED_EDGE ( 'NONE', *, *, #119741, .F. ) ;
#59706=DIRECTION ( 'NONE',  ( 0.000000000000000000, -0.9999939076577903929, 0.003490651415223739937 ) ) ;
#59707=EDGE_LOOP ( 'NONE', ( #16567, #28715 ) ) ;
#59708=CARTESIAN_POINT ( 'NONE',  ( 17.50000000000010658, -2.262047038896518369, 3.993694673355226321 ) ) ;
#59709=CARTESIAN_POINT ( 'NONE',  ( 11.24999999999990585, 2.500000000000000000, 2.857883832488649301 ) ) ;
#59710=AXIS2_PLACEMENT_3D ( 'NONE', #11633, #41763, #111096 ) ;
#59711=ORIENTED_EDGE ( 'NONE', *, *, #108203, .T. ) ;
#59712=CARTESIAN_POINT ( 'NONE',  ( 0.6499999999999561684, 2.500000000000000000, -2.511473670974877948 ) ) ;
#59713=DIRECTION ( 'NONE',  ( 0.000000000000000000, 0.000000000000000000, -1.000000000000000000 ) ) ;
#59714=CARTESIAN_POINT ( 'NONE',  ( 5.449999999999936229, 12.50000000000000000, -2.165063509461101710 ) ) ;
#59715=AXIS2_PLACEMENT_3D ( 'NONE', #96164, #88936, #88262 ) ;
#59716=FACE_OUTER_BOUND ( 'NONE', #75704, .T. ) ;
#59717=CIRCLE ( 'NONE', #95383, 0.06509327318403745899 ) ;
#59718=DIRECTION ( 'NONE',  ( 0.000000000000000000, 1.000000000000000000, 0.000000000000000000 ) ) ;
#59719=AXIS2_PLACEMENT_3D ( 'NONE', #99114, #43432, #2181 ) ;
#59720=ORIENTED_EDGE ( 'NONE', *, *, #86683, .T. ) ;
#59721=CARTESIAN_POINT ( 'NONE',  ( -8.750000000000008882, 2.500000000000000000, -2.957883832488653830 ) ) ;
#59722=DIRECTION ( 'NONE',  ( 0.000000000000000000, 0.000000000000000000, 1.000000000000000000 ) ) ;
#59723=DIRECTION ( 'NONE',  ( -4.274815082592931898E-19, -0.9999939076577903929, -0.003490651415223739937 ) ) ;
#59724=AXIS2_PLACEMENT_3D ( 'NONE', #117908, #28252, #68165 ) ;
#59725=VERTEX_POINT ( 'NONE', #113815 ) ;
#59726=CARTESIAN_POINT ( 'NONE',  ( -10.60000000000000142, 2.500000000000000000, 4.676537180435972552 ) ) ;
#59727=EDGE_CURVE ( 'NONE', #56812, #63511, #91593, .T. ) ;
#59728=AXIS2_PLACEMENT_3D ( 'NONE', #103140, #43600, #123417 ) ;
#59729=ORIENTED_EDGE ( 'NONE', *, *, #68527, .T. ) ;
#59730=DIRECTION ( 'NONE',  ( -4.274815082592931898E-19, -0.9999939076577903929, -0.003490651415223739937 ) ) ;
#59731=DIRECTION ( 'NONE',  ( 0.000000000000000000, 1.000000000000000000, 0.000000000000000000 ) ) ;
#59732=CARTESIAN_POINT ( 'NONE',  ( 3.749999999999942268, 2.500000000000000000, -1.372243186433550033 ) ) ;
#59733=VERTEX_POINT ( 'NONE', #73242 ) ;
#59734=AXIS2_PLACEMENT_3D ( 'NONE', #108900, #110842, #90563 ) ;
#59735=CIRCLE ( 'NONE', #53459, 0.06509327318403745899 ) ;
#59736=DIRECTION ( 'NONE',  ( 0.000000000000000000, 0.000000000000000000, -1.000000000000000000 ) ) ;
#59737=AXIS2_PLACEMENT_3D ( 'NONE', #117374, #79435, #41451 ) ;
#59738=CARTESIAN_POINT ( 'NONE',  ( -3.350000000000028511, 2.500000000000000000, -2.857883832488653741 ) ) ;
#59739=AXIS2_PLACEMENT_3D ( 'NONE', #114547, #55644, #45193 ) ;
#59740=EDGE_CURVE ( 'NONE', #120245, #66596, #67864, .T. ) ;
#59741=EDGE_LOOP ( 'NONE', ( #9676, #62025 ) ) ;
#59742=CARTESIAN_POINT ( 'NONE',  ( -10.60000000000000142, 12.50000000000000000, 4.676537180435972552 ) ) ;
#59743=EDGE_CURVE ( 'NONE', #58412, #85724, #124306, .T. ) ;
#59744=EDGE_LOOP ( 'NONE', ( #118239, #81633 ) ) ;
#59745=FACE_OUTER_BOUND ( 'NONE', #66502, .T. ) ;
#59746=ORIENTED_EDGE ( 'NONE', *, *, #81631, .T. ) ;
#59747=DIRECTION ( 'NONE',  ( 0.000000000000000000, 1.000000000000000000, 0.000000000000000000 ) ) ;
#59748=DIRECTION ( 'NONE',  ( 0.000000000000000000, 0.000000000000000000, 1.000000000000000000 ) ) ;
#59749=ORIENTED_EDGE ( 'NONE', *, *, #1697, .T. ) ;
#59750=EDGE_CURVE ( 'NONE', #59274, #17587, #99183, .T. ) ;
#59751=EDGE_LOOP ( 'NONE', ( #121423, #58746 ) ) ;
#59752=DIRECTION ( 'NONE',  ( -0.000000000000000000, 1.000000000000000000, -0.000000000000000000 ) ) ;
#59753=DIRECTION ( 'NONE',  ( -0.000000000000000000, 1.000000000000000000, -0.000000000000000000 ) ) ;
#59754=CIRCLE ( 'NONE', #17859, 0.06509327318403745899 ) ;
#59755=ORIENTED_EDGE ( 'NONE', *, *, #26387, .F. ) ;
#59756=DIRECTION ( 'NONE',  ( -0.000000000000000000, 1.000000000000000000, -0.000000000000000000 ) ) ;
#59758=CARTESIAN_POINT ( 'NONE',  ( -2.499999999999996447, 2.500000000000000000, 4.330127018922196314 ) ) ;
#59759=CARTESIAN_POINT ( 'NONE',  ( 9.349999999999916156, 2.500000000000000000, -2.611473670974877592 ) ) ;
#59760=CARTESIAN_POINT ( 'NONE',  ( 9.149999999999916866, 2.500000000000000000, -2.957883832488653830 ) ) ;
#59761=FACE_OUTER_BOUND ( 'NONE', #115968, .T. ) ;
#59762=CIRCLE ( 'NONE', #13750, 0.1000000000000002554 ) ;
#59763=FACE_OUTER_BOUND ( 'NONE', #110314, .T. ) ;
#59764=CIRCLE ( 'NONE', #36774, 0.06509327318403745899 ) ;
#59765=VECTOR ( 'NONE', #52014, 1000.000000000000000 ) ;
#59766=ORIENTED_EDGE ( 'NONE', *, *, #125101, .T. ) ;
#59767=EDGE_CURVE ( 'NONE', #73054, #60265, #63682, .T. ) ;
#59768=ORIENTED_EDGE ( 'NONE', *, *, #50922, .T. ) ;
#59769=ORIENTED_EDGE ( 'NONE', *, *, #4004, .F. ) ;
#59770=ORIENTED_EDGE ( 'NONE', *, *, #17863, .F. ) ;
#59771=B_SPLINE_CURVE_WITH_KNOTS ( 'NONE', 3,
 ( #32964, #64962, #33595, #44050 ),
 .UNSPECIFIED., .F., .F.,
 ( 4, 4 ),
 ( 0.2000000000000000666, 0.7999999999999999334 ),
 .UNSPECIFIED. ) ;
#59772=DIRECTION ( 'NONE',  ( 0.000000000000000000, 1.000000000000000000, 0.000000000000000000 ) ) ;
#59773=CARTESIAN_POINT ( 'NONE',  ( 6.649999999999930189, 12.50000000000000000, 5.737276932171707422 ) ) ;
#59774=DIRECTION ( 'NONE',  ( -0.000000000000000000, 1.000000000000000000, -0.000000000000000000 ) ) ;
#59775=ORIENTED_EDGE ( 'NONE', *, *, #60518, .F. ) ;
#59776=FACE_BOUND ( 'NONE', #64525, .T. ) ;
#59777=EDGE_LOOP ( 'NONE', ( #53812, #93269 ) ) ;
#59778=DIRECTION ( 'NONE',  ( 0.000000000000000000, 1.000000000000000000, 0.000000000000000000 ) ) ;
#59779=CARTESIAN_POINT ( 'NONE',  ( -0.4000000000000396572, 12.50000000000000000, 4.330127018922196314 ) ) ;
#59780=CARTESIAN_POINT ( 'NONE',  ( 9.149999999999920419, 2.500000000000000000, -5.802370205355749988 ) ) ;
#59781=ADVANCED_FACE ( 'NONE', ( #122355 ), #111882, .T. ) ;
#59782=DIRECTION ( 'NONE',  ( -0.000000000000000000, -1.000000000000000000, -0.000000000000000000 ) ) ;
#59783=AXIS2_PLACEMENT_3D ( 'NONE', #106137, #5982, #85837 ) ;
#59784=VECTOR ( 'NONE', #23698, 1000.000000000000000 ) ;
#59785=CARTESIAN_POINT ( 'NONE',  ( -15.59999999999998010, 2.500000000000000000, -0.3464101615137759604 ) ) ;
#59786=CARTESIAN_POINT ( 'NONE',  ( 1.849999999999950573, 12.50000000000000000, -1.883746621131363597 ) ) ;
#59787=DIRECTION ( 'NONE',  ( 0.000000000000000000, 0.000000000000000000, 1.000000000000000000 ) ) ;
#59788=FACE_OUTER_BOUND ( 'NONE', #40836, .T. ) ;
#59789=EDGE_CURVE ( 'NONE', #80777, #84307, #102063, .T. ) ;
#59790=EDGE_CURVE ( 'NONE', #52044, #127925, #52313, .T. ) ;
#59791=DIRECTION ( 'NONE',  ( 0.000000000000000000, 0.000000000000000000, -1.000000000000000000 ) ) ;
#59792=EDGE_CURVE ( 'NONE', #72896, #75229, #22872, .T. ) ;
#59793=EDGE_CURVE ( 'NONE', #88292, #48784, #122992, .T. ) ;
#59794=DIRECTION ( 'NONE',  ( 0.000000000000000000, 1.000000000000000000, 0.000000000000000000 ) ) ;
#59795=CIRCLE ( 'NONE', #49324, 0.06509327318403745899 ) ;
#59796=ORIENTED_EDGE ( 'NONE', *, *, #12716, .T. ) ;
#59797=VERTEX_POINT ( 'NONE', #83714 ) ;
#59798=CIRCLE ( 'NONE', #80708, 0.1000000000000002554 ) ;
#59799=EDGE_LOOP ( 'NONE', ( #62337, #71892 ) ) ;
#59800=ORIENTED_EDGE ( 'NONE', *, *, #80513, .F. ) ;
#59801=PLANE ( 'NONE',  #106407 ) ;
#59802=EDGE_CURVE ( 'NONE', #69160, #62906, #42773, .T. ) ;
#59803=DIRECTION ( 'NONE',  ( 0.000000000000000000, 0.000000000000000000, 1.000000000000000000 ) ) ;
#59804=EDGE_CURVE ( 'NONE', #97882, #22999, #86260, .T. ) ;
#59805=ORIENTED_EDGE ( 'NONE', *, *, #71190, .T. ) ;
#59806=EDGE_LOOP ( 'NONE', ( #118303, #6368 ) ) ;
#59807=ORIENTED_EDGE ( 'NONE', *, *, #10283, .F. ) ;
#59808=CARTESIAN_POINT ( 'NONE',  ( 10.84999999999990905, 2.500000000000000000, -7.288010851410854585 ) ) ;
#59809=ADVANCED_FACE ( 'NONE', ( #57476 ), #74532, .T. ) ;
#59810=ADVANCED_FACE ( 'NONE', ( #36559 ), #35266, .T. ) ;
#59811=FACE_OUTER_BOUND ( 'NONE', #15827, .T. ) ;
#59812=DIRECTION ( 'NONE',  ( -4.274815082592931898E-19, -0.9999939076577903929, -0.003490651415223739937 ) ) ;
#59813=DIRECTION ( 'NONE',  ( 0.000000000000000000, 1.000000000000000000, 0.000000000000000000 ) ) ;
#59814=CARTESIAN_POINT ( 'NONE',  ( 6.649999999999930189, 2.500000000000000000, 7.288010851410849256 ) ) ;
#59815=CARTESIAN_POINT ( 'NONE',  ( 2.500000000000002220, 1.761799387799150018, 10.00000000000000000 ) ) ;
#59816=CARTESIAN_POINT ( 'NONE',  ( 7.099999999999928590, 2.500000000000000000, 3.637306695894644726 ) ) ;
#59817=ADVANCED_FACE ( 'NONE', ( #76471 ), #16227, .T. ) ;
#59818=ORIENTED_EDGE ( 'NONE', *, *, #43814, .T. ) ;
#59819=ADVANCED_FACE ( 'NONE', ( #5134 ), #27338, .T. ) ;
#59820=DIRECTION ( 'NONE',  ( 0.000000000000000000, 1.000000000000000000, 0.000000000000000000 ) ) ;
#59821=ORIENTED_EDGE ( 'NONE', *, *, #25748, .T. ) ;
#59822=AXIS2_PLACEMENT_3D ( 'NONE', #119972, #30323, #100337 ) ;
#59823=EDGE_LOOP ( 'NONE', ( #61000, #45183 ) ) ;
#59824=ORIENTED_EDGE ( 'NONE', *, *, #46181, .F. ) ;
#59825=AXIS2_PLACEMENT_3D ( 'NONE', #19756, #117934, #89128 ) ;
#59826=DIRECTION ( 'NONE',  ( -0.000000000000000000, -1.000000000000000000, -0.000000000000000000 ) ) ;
#59827=ORIENTED_EDGE ( 'NONE', *, *, #27522, .T. ) ;
#59828=EDGE_LOOP ( 'NONE', ( #25771, #52344, #4446, #110769 ) ) ;
#59829=DIRECTION ( 'NONE',  ( 0.000000000000000000, 0.000000000000000000, -1.000000000000000000 ) ) ;
#59830=AXIS2_PLACEMENT_3D ( 'NONE', #66631, #98666, #7059 ) ;
#59831=FACE_OUTER_BOUND ( 'NONE', #109723, .T. ) ;
#59832=CARTESIAN_POINT ( 'NONE',  ( -15.39999999999997904, 2.500000000000000000, 0.000000000000000000 ) ) ;
#59833=DIRECTION ( 'NONE',  ( -0.000000000000000000, -1.000000000000000000, -0.000000000000000000 ) ) ;
#59834=PLANE ( 'NONE',  #56656 ) ;
#59836=DIRECTION ( 'NONE',  ( 0.000000000000000000, 0.000000000000000000, -1.000000000000000000 ) ) ;
#59837=CIRCLE ( 'NONE', #45232, 0.1000000000000002554 ) ;
#59838=EDGE_LOOP ( 'NONE', ( #61003, #61481 ) ) ;
#59839=CARTESIAN_POINT ( 'NONE',  ( 18.45986577996939104, -0.7763546025154367536, 4.045836809868020190 ) ) ;
#59840=AXIS2_PLACEMENT_3D ( 'NONE', #95690, #8564, #48517 ) ;
#59841=ORIENTED_EDGE ( 'NONE', *, *, #51437, .F. ) ;
#59842=FACE_OUTER_BOUND ( 'NONE', #117670, .T. ) ;
#59843=PLANE ( 'NONE',  #1017 ) ;
#59844=VERTEX_POINT ( 'NONE', #45084 ) ;
#59845=DIRECTION ( 'NONE',  ( -0.000000000000000000, 1.000000000000000000, -0.000000000000000000 ) ) ;
#59846=FACE_OUTER_BOUND ( 'NONE', #76640, .T. ) ;
#59847=EDGE_LOOP ( 'NONE', ( #70788, #48279, #53420, #56858 ) ) ;
#59848=ADVANCED_FACE ( 'NONE', ( #84982 ), #11434, .T. ) ;
#59849=DIRECTION ( 'NONE',  ( 0.000000000000000000, 0.000000000000000000, 1.000000000000000000 ) ) ;
#59850=EDGE_CURVE ( 'NONE', #64883, #112256, #17685, .T. ) ;
#59851=ORIENTED_EDGE ( 'NONE', *, *, #69047, .F. ) ;
#59852=VERTEX_POINT ( 'NONE', #96097 ) ;
#59853=DIRECTION ( 'NONE',  ( 0.000000000000000000, -0.000000000000000000, 1.000000000000000000 ) ) ;
#59854=CARTESIAN_POINT ( 'NONE',  ( 8.949999999999921130, 12.50000000000000000, 1.883746621131358934 ) ) ;
#59855=DIRECTION ( 'NONE',  ( -4.274815082592931898E-19, -0.9999939076577903929, -0.003490651415223739937 ) ) ;
#59856=AXIS2_PLACEMENT_3D ( 'NONE', #84382, #44457, #56200 ) ;
#59857=CARTESIAN_POINT ( 'NONE',  ( -5.600000000000023626, 2.500000000000000000, -4.576537180435977348 ) ) ;
#59858=DIRECTION ( 'NONE',  ( 0.000000000000000000, 0.000000000000000000, 1.000000000000000000 ) ) ;
#59859=EDGE_LOOP ( 'NONE', ( #105182, #113775, #94385, #85373 ) ) ;
#59860=AXIS2_PLACEMENT_3D ( 'NONE', #44511, #37916, #117100 ) ;
#59861=FACE_OUTER_BOUND ( 'NONE', #70929, .T. ) ;
#59862=AXIS2_PLACEMENT_3D ( 'NONE', #91473, #100637, #81651 ) ;
#59863=CIRCLE ( 'NONE', #51525, 0.09999999999999999167 ) ;
#59864=ORIENTED_EDGE ( 'NONE', *, *, #53265, .T. ) ;
#59865=AXIS2_PLACEMENT_3D ( 'NONE', #91769, #23035, #121229 ) ;
#59866=DIRECTION ( 'NONE',  ( 0.000000000000000000, 0.000000000000000000, 1.000000000000000000 ) ) ;
#59867=DIRECTION ( 'NONE',  ( 0.000000000000000000, -0.9999939076577903929, 0.003490651415223739937 ) ) ;
#59868=CIRCLE ( 'NONE', #109927, 0.06509327318403745899 ) ;
#59870=CARTESIAN_POINT ( 'NONE',  ( 9.349999999999919709, 2.500000000000000000, -6.741600689897078169 ) ) ;
#59871=FACE_OUTER_BOUND ( 'NONE', #121344, .T. ) ;
#59874=ORIENTED_EDGE ( 'NONE', *, *, #27834, .F. ) ;
#59875=CIRCLE ( 'NONE', #5445, 0.06509327318403745899 ) ;
#59876=DIRECTION ( 'NONE',  ( 0.000000000000000000, 0.000000000000000000, -1.000000000000000000 ) ) ;
#59877=CONICAL_SURFACE ( 'NONE', #105816, 0.1000000000000002554, 0.003490658503988666988 ) ;
#59878=CIRCLE ( 'NONE', #76577, 0.1000000000000002554 ) ;
#59879=DIRECTION ( 'NONE',  ( 0.000000000000000000, 0.000000000000000000, 1.000000000000000000 ) ) ;
#59880=DIRECTION ( 'NONE',  ( -0.000000000000000000, 1.000000000000000000, -0.000000000000000000 ) ) ;
#59881=ORIENTED_EDGE ( 'NONE', *, *, #105700, .F. ) ;
#59882=DIRECTION ( 'NONE',  ( 0.000000000000000000, 0.000000000000000000, -1.000000000000000000 ) ) ;
#59883=ADVANCED_FACE ( 'NONE', ( #16858 ), #61628, .T. ) ;
#59884=VERTEX_POINT ( 'NONE', #25407 ) ;
#59885=ORIENTED_EDGE ( 'NONE', *, *, #129392, .F. ) ;
#59886=CARTESIAN_POINT ( 'NONE',  ( 3.549999999999942091, 12.50000000000000000, 2.576566944158910744 ) ) ;
#59887=ORIENTED_EDGE ( 'NONE', *, *, #6803, .T. ) ;
#59888=DIRECTION ( 'NONE',  ( 0.000000000000000000, 1.000000000000000000, 0.000000000000000000 ) ) ;
#59889=CARTESIAN_POINT ( 'NONE',  ( 8.149999999999923972, 2.500000000000000000, -6.941600689897077459 ) ) ;
#59890=ORIENTED_EDGE ( 'NONE', *, *, #9857, .F. ) ;
#59891=PLANE ( 'NONE',  #88535 ) ;
#59892=CARTESIAN_POINT ( 'NONE',  ( 3.749999999999938716, 2.500000000000000000, 7.188010851410848723 ) ) ;
#59893=EDGE_CURVE ( 'NONE', #137, #115201, #118042, .T. ) ;
#59894=DIRECTION ( 'NONE',  ( 0.000000000000000000, 1.000000000000000000, 0.000000000000000000 ) ) ;
#59895=EDGE_CURVE ( 'NONE', #124839, #24998, #55353, .T. ) ;
#59896=EDGE_LOOP ( 'NONE', ( #110813, #102259 ) ) ;
#59897=VECTOR ( 'NONE', #24197, 1000.000000000000000 ) ;
#59898=EDGE_LOOP ( 'NONE', ( #38917, #83992, #19454, #100031 ) ) ;
#59900=ORIENTED_EDGE ( 'NONE', *, *, #125665, .F. ) ;
#59901=DIRECTION ( 'NONE',  ( 0.000000000000000000, 0.000000000000000000, 1.000000000000000000 ) ) ;
#59902=DIRECTION ( 'NONE',  ( 0.000000000000000000, -0.9999939076577903929, 0.003490651415223739937 ) ) ;
#59903=CARTESIAN_POINT ( 'NONE',  ( -8.750000000000008882, 2.500000000000000000, 1.572243186433545548 ) ) ;
#59904=EDGE_CURVE ( 'NONE', #72819, #85157, #64701, .T. ) ;
#59905=FACE_BOUND ( 'NONE', #73461, .T. ) ;
#59907=DIRECTION ( 'NONE',  ( -0.000000000000000000, 1.000000000000000000, -0.000000000000000000 ) ) ;
#59908=CARTESIAN_POINT ( 'NONE',  ( -3.749999999999991118, 12.50000000000000000, -2.165063509461101710 ) ) ;
#59909=EDGE_LOOP ( 'NONE', ( #128421, #11689, #35598, #120128 ) ) ;
#59910=AXIS2_PLACEMENT_3D ( 'NONE', #100261, #89141, #21042 ) ;
#59911=CIRCLE ( 'NONE', #80738, 0.09999999999999999167 ) ;
#59912=DIRECTION ( 'NONE',  ( 0.000000000000000000, 0.000000000000000000, 1.000000000000000000 ) ) ;
#59913=DIRECTION ( 'NONE',  ( 0.000000000000000000, -0.000000000000000000, 1.000000000000000000 ) ) ;
#59914=DIRECTION ( 'NONE',  ( -0.000000000000000000, -1.000000000000000000, -0.000000000000000000 ) ) ;
#59915=PLANE ( 'NONE',  #36143 ) ;
#59916=CARTESIAN_POINT ( 'NONE',  ( -2.499999999999996003, 12.50000000000000000, -2.276824562219559311E-15 ) ) ;
#59917=CARTESIAN_POINT ( 'NONE',  ( 11.24999999999990585, 12.50000000000000000, 2.857883832488649301 ) ) ;
#59918=CARTESIAN_POINT ( 'NONE',  ( 11.84999999999990372, 2.500000000000000000, -6.048780366869526581 ) ) ;
#59919=AXIS2_PLACEMENT_3D ( 'NONE', #91706, #53070, #43269 ) ;
#59920=VECTOR ( 'NONE', #91747, 1000.000000000000000 ) ;
#59921=AXIS2_PLACEMENT_3D ( 'NONE', #111274, #61575, #101489 ) ;
#59922=ORIENTED_EDGE ( 'NONE', *, *, #72617, .T. ) ;
#59923=ORIENTED_EDGE ( 'NONE', *, *, #91159, .F. ) ;
#59924=ORIENTED_EDGE ( 'NONE', *, *, #7565, .T. ) ;
#59925=ORIENTED_EDGE ( 'NONE', *, *, #87927, .F. ) ;
#59926=ORIENTED_EDGE ( 'NONE', *, *, #128472, .F. ) ;
#59927=CARTESIAN_POINT ( 'NONE',  ( 13.54999999999990123, 2.500000000000000000, 1.818653347947321475 ) ) ;
#59928=LINE ( 'NONE', #88039, #124055 ) ;
#59929=EDGE_LOOP ( 'NONE', ( #50880, #29393 ) ) ;
#59930=FACE_BOUND ( 'NONE', #74795, .T. ) ;
#59931=DIRECTION ( 'NONE',  ( 0.000000000000000000, 0.000000000000000000, 1.000000000000000000 ) ) ;
#59932=EDGE_CURVE ( 'NONE', #111598, #3394, #63768, .T. ) ;
#59933=CARTESIAN_POINT ( 'NONE',  ( -1.700000000000034817, 2.500000000000000000, -4.430127018922202176 ) ) ;
#59934=CARTESIAN_POINT ( 'NONE',  ( -10.85000000000000142, 12.50000000000000000, -6.495190528383298911 ) ) ;
#59936=DIRECTION ( 'NONE',  ( -0.000000000000000000, -1.000000000000000000, -0.000000000000000000 ) ) ;
#59937=EDGE_CURVE ( 'NONE', #81531, #59613, #65335, .T. ) ;
#59938=DIRECTION ( 'NONE',  ( 0.000000000000000000, 0.000000000000000000, -1.000000000000000000 ) ) ;
#59939=AXIS2_PLACEMENT_3D ( 'NONE', #5163, #45114, #85019 ) ;
#59940=VERTEX_POINT ( 'NONE', #125551 ) ;
#59941=EDGE_CURVE ( 'NONE', #45135, #77998, #82558, .T. ) ;
#59942=AXIS2_PLACEMENT_3D ( 'NONE', #118028, #68928, #8072 ) ;
#59943=EDGE_LOOP ( 'NONE', ( #54795, #114518 ) ) ;
#59944=EDGE_LOOP ( 'NONE', ( #127699, #46821 ) ) ;
#59945=VECTOR ( 'NONE', #37011, 1000.000000000000000 ) ;
#59946=VERTEX_POINT ( 'NONE', #15594 ) ;
#59947=ORIENTED_EDGE ( 'NONE', *, *, #64339, .T. ) ;
#59948=VERTEX_POINT ( 'NONE', #75803 ) ;
#59949=EDGE_CURVE ( 'NONE', #123441, #100484, #22016, .T. ) ;
#59951=ADVANCED_FACE ( 'NONE', ( #47017 ), #3133, .T. ) ;
#59952=CARTESIAN_POINT ( 'NONE',  ( 6.249999999999967137, 12.50000000000000000, 6.560283801567334372 ) ) ;
#59953=EDGE_CURVE ( 'NONE', #114987, #40225, #40425, .T. ) ;
#59954=VERTEX_POINT ( 'NONE', #58124 ) ;
#59955=CARTESIAN_POINT ( 'NONE',  ( 4.599999999999939249, 12.50000000000000000, -3.637306695894650055 ) ) ;
#59956=VECTOR ( 'NONE', #15105, 1000.000000000000000 ) ;
#59957=AXIS2_PLACEMENT_3D ( 'NONE', #29327, #40447, #50897 ) ;
#59958=DIRECTION ( 'NONE',  ( 0.000000000000000000, 0.000000000000000000, 1.000000000000000000 ) ) ;
#59959=CIRCLE ( 'NONE', #3493, 0.1000000000000002554 ) ;
#59960=PLANE ( 'NONE',  #78807 ) ;
#59961=ADVANCED_FACE ( 'NONE', ( #117644 ), #115988, .T. ) ;
#59963=DIRECTION ( 'NONE',  ( 0.000000000000000000, 0.000000000000000000, -1.000000000000000000 ) ) ;
#59964=CARTESIAN_POINT ( 'NONE',  ( -5.650000000000023448, 12.50000000000000000, -2.446380397790840266 ) ) ;
#59965=DIRECTION ( 'NONE',  ( -0.000000000000000000, 1.000000000000000000, -0.000000000000000000 ) ) ;
#59966=CONICAL_SURFACE ( 'NONE', #51628, 0.1000000000000002554, 0.003490658503988666988 ) ;
#59967=EDGE_LOOP ( 'NONE', ( #59775, #69911, #55485, #93746 ) ) ;
#59968=FACE_OUTER_BOUND ( 'NONE', #103787, .T. ) ;
#59969=EDGE_CURVE ( 'NONE', #32170, #70149, #7311, .T. ) ;
#59970=AXIS2_PLACEMENT_3D ( 'NONE', #126532, #28981, #38148 ) ;
#59972=CIRCLE ( 'NONE', #124782, 0.1000000000000002554 ) ;
#59973=AXIS2_PLACEMENT_3D ( 'NONE', #25446, #94858, #16898 ) ;
#59974=ORIENTED_EDGE ( 'NONE', *, *, #92511, .F. ) ;
#59975=DIRECTION ( 'NONE',  ( 0.000000000000000000, 0.000000000000000000, -1.000000000000000000 ) ) ;
#59976=DIRECTION ( 'NONE',  ( -0.000000000000000000, -1.000000000000000000, -0.000000000000000000 ) ) ;
#59977=FACE_OUTER_BOUND ( 'NONE', #126977, .T. ) ;
#59978=EDGE_LOOP ( 'NONE', ( #37238, #58022, #103460, #89964 ) ) ;
#59979=EDGE_LOOP ( 'NONE', ( #125862, #106286, #84666, #124976 ) ) ;
#59980=DIRECTION ( 'NONE',  ( 0.000000000000000000, 1.000000000000000000, 0.000000000000000000 ) ) ;
#59981=DIRECTION ( 'NONE',  ( -0.000000000000000000, 1.000000000000000000, -0.000000000000000000 ) ) ;
#59982=FACE_OUTER_BOUND ( 'NONE', #113549, .T. ) ;
#59983=DIRECTION ( 'NONE',  ( 0.000000000000000000, 0.000000000000000000, 1.000000000000000000 ) ) ;
#59984=ORIENTED_EDGE ( 'NONE', *, *, #21441, .F. ) ;
#59985=DIRECTION ( 'NONE',  ( -0.000000000000000000, 1.000000000000000000, -0.000000000000000000 ) ) ;
#59986=CIRCLE ( 'NONE', #114412, 0.1000000000000000056 ) ;
#59987=ORIENTED_EDGE ( 'NONE', *, *, #107531, .F. ) ;
#59988=LINE ( 'NONE', #38407, #68738 ) ;
#59989=VERTEX_POINT ( 'NONE', #28664 ) ;
#59990=DIRECTION ( 'NONE',  ( 0.000000000000000000, 0.000000000000000000, -1.000000000000000000 ) ) ;
#59991=DIRECTION ( 'NONE',  ( -0.000000000000000000, 1.000000000000000000, -0.000000000000000000 ) ) ;
#59992=CARTESIAN_POINT ( 'NONE',  ( 10.44999999999991047, 12.50000000000000000, 2.230156782645134950 ) ) ;
#59993=DIRECTION ( 'NONE',  ( -0.000000000000000000, 1.000000000000000000, -0.000000000000000000 ) ) ;
#59994=ORIENTED_EDGE ( 'NONE', *, *, #17941, .T. ) ;
#59995=DIRECTION ( 'NONE',  ( 0.000000000000000000, 0.000000000000000000, 1.000000000000000000 ) ) ;
#59997=EDGE_CURVE ( 'NONE', #105793, #15915, #120265, .T. ) ;
#59998=ORIENTED_EDGE ( 'NONE', *, *, #114763, .T. ) ;
#59999=ORIENTED_EDGE ( 'NONE', *, *, #57819, .T. ) ;
#60000=CARTESIAN_POINT ( 'NONE',  ( -1.650000000000034328, 2.500000000000000000, -2.957883832488653830 ) ) ;
#60001=CARTESIAN_POINT ( 'NONE',  ( 5.799999999999933209, 2.500000000000000000, -2.385244779468109755E-15 ) ) ;
#60002=PLANE ( 'NONE',  #32389 ) ;
#60004=FACE_OUTER_BOUND ( 'NONE', #11020, .T. ) ;
#60005=CONICAL_SURFACE ( 'NONE', #95479, 0.1000000000000000472, 0.003490658503988666988 ) ;
#60006=DIRECTION ( 'NONE',  ( 0.000000000000000000, 0.000000000000000000, 1.000000000000000000 ) ) ;
#60007=CONICAL_SURFACE ( 'NONE', #32808, 0.09999999999999982514, 0.003490658503988666988 ) ;
#60008=ADVANCED_FACE ( 'NONE', ( #39782 ), #109738, .T. ) ;
#60009=DIRECTION ( 'NONE',  ( -0.000000000000000000, 1.000000000000000000, -0.000000000000000000 ) ) ;
#60010=CARTESIAN_POINT ( 'NONE',  ( -10.85000000000000142, 2.500000000000000000, 2.265063509461097357 ) ) ;
#60011=CARTESIAN_POINT ( 'NONE',  ( 6.449999999999928235, 2.500000000000000000, 2.611473670974873151 ) ) ;
#60012=CIRCLE ( 'NONE', #101844, 0.1000000000000002554 ) ;
#60013=CIRCLE ( 'NONE', #108004, 0.09999999999999982514 ) ;
#60014=AXIS2_PLACEMENT_3D ( 'NONE', #59927, #6901, #46867 ) ;
#60015=EDGE_LOOP ( 'NONE', ( #57887, #40758 ) ) ;
#60016=CARTESIAN_POINT ( 'NONE',  ( 13.54999999999989591, 12.50000000000000000, -1.883746621131363597 ) ) ;
#60017=DIRECTION ( 'NONE',  ( -0.000000000000000000, 1.000000000000000000, -0.000000000000000000 ) ) ;
#60018=DIRECTION ( 'NONE',  ( 0.000000000000000000, 0.000000000000000000, 1.000000000000000000 ) ) ;
#60019=CARTESIAN_POINT ( 'NONE',  ( -3.100000000000028511, 2.500000000000000000, -4.576537180435977348 ) ) ;
#60020=FACE_OUTER_BOUND ( 'NONE', #98826, .T. ) ;
#60021=VERTEX_POINT ( 'NONE', #98031 ) ;
#60022=DIRECTION ( 'NONE',  ( 0.000000000000000000, -0.9999939076577903929, 0.003490651415223739937 ) ) ;
#60023=CARTESIAN_POINT ( 'NONE',  ( -7.700000000000012612, 2.500000000000000000, 4.676537180435972552 ) ) ;
#60024=DIRECTION ( 'NONE',  ( 0.000000000000000000, -0.9999939076577903929, 0.003490651415223739937 ) ) ;
#60025=EDGE_LOOP ( 'NONE', ( #106561, #97370, #115746, #129580 ) ) ;
#60026=VECTOR ( 'NONE', #100175, 1000.000000000000000 ) ;
#60027=VERTEX_POINT ( 'NONE', #129462 ) ;
#60028=CARTESIAN_POINT ( 'NONE',  ( 6.849999999999927702, 2.500000000000000000, 1.918653347947321564 ) ) ;
#60029=EDGE_CURVE ( 'NONE', #56111, #53781, #113940, .T. ) ;
#60030=CIRCLE ( 'NONE', #30784, 0.1000000000000000056 ) ;
#60031=ORIENTED_EDGE ( 'NONE', *, *, #129287, .F. ) ;
#60032=ORIENTED_EDGE ( 'NONE', *, *, #86361, .T. ) ;
#60033=CARTESIAN_POINT ( 'NONE',  ( 7.899999999999924860, 12.50000000000000000, 3.637306695894644726 ) ) ;
#60034=AXIS2_PLACEMENT_3D ( 'NONE', #124131, #52816, #23339 ) ;
#60035=DIRECTION ( 'NONE',  ( 0.000000000000000000, 1.000000000000000000, 0.000000000000000000 ) ) ;
#60036=CARTESIAN_POINT ( 'NONE',  ( 13.14999999999989733, 2.500000000000000000, -2.611473670974877592 ) ) ;
#60037=VECTOR ( 'NONE', #102554, 1000.000000000000000 ) ;
#60038=DIRECTION ( 'NONE',  ( 0.000000000000000000, 0.000000000000000000, 1.000000000000000000 ) ) ;
#60039=EDGE_CURVE ( 'NONE', #35443, #114904, #67952, .T. ) ;
#60040=VERTEX_POINT ( 'NONE', #454 ) ;
#60041=CARTESIAN_POINT ( 'NONE',  ( 13.74999999999993427, 12.50000000000000000, 2.165063509461097713 ) ) ;
#60042=EDGE_LOOP ( 'NONE', ( #101274, #88325 ) ) ;
#60043=CARTESIAN_POINT ( 'NONE',  ( 8.749999999999957367, 12.50000000000000000, -6.495190528383302464 ) ) ;
#60044=EDGE_CURVE ( 'NONE', #27533, #29548, #49601, .T. ) ;
#60045=CARTESIAN_POINT ( 'NONE',  ( -5.800000000000022027, 12.50000000000000000, -4.330127018922201643 ) ) ;
#60046=AXIS2_PLACEMENT_3D ( 'NONE', #98088, #59492, #8406 ) ;
#60047=DIRECTION ( 'NONE',  ( 0.000000000000000000, 0.000000000000000000, -1.000000000000000000 ) ) ;
#60048=EDGE_CURVE ( 'NONE', #117860, #109761, #42863, .T. ) ;
#60049=CONICAL_SURFACE ( 'NONE', #62099, 0.1000000000000002554, 0.003490658503988666988 ) ;
#60050=EDGE_LOOP ( 'NONE', ( #128366, #94479, #11825, #53223 ) ) ;
#60051=ORIENTED_EDGE ( 'NONE', *, *, #57397, .F. ) ;
#60052=EDGE_CURVE ( 'NONE', #128668, #53584, #57504, .T. ) ;
#60053=ORIENTED_EDGE ( 'NONE', *, *, #118244, .T. ) ;
#60054=ORIENTED_EDGE ( 'NONE', *, *, #122595, .F. ) ;
#60055=ORIENTED_EDGE ( 'NONE', *, *, #76454, .T. ) ;
#60056=DIRECTION ( 'NONE',  ( -0.000000000000000000, 1.000000000000000000, -0.000000000000000000 ) ) ;
#60057=CARTESIAN_POINT ( 'NONE',  ( 15.62882261213669999, 2.499999999999999556, 5.624357572923773141 ) ) ;
#60058=DIRECTION ( 'NONE',  ( 0.000000000000000000, 0.000000000000000000, -1.000000000000000000 ) ) ;
#60059=EDGE_CURVE ( 'NONE', #104314, #19521, #30337, .T. ) ;
#60060=FACE_BOUND ( 'NONE', #1329, .T. ) ;
#60061=CARTESIAN_POINT ( 'NONE',  ( 11.64999999999990443, 2.500000000000000000, 1.372243186433545370 ) ) ;
#60063=CARTESIAN_POINT ( 'NONE',  ( 10.84999999999991260, 2.500000000000000000, -2.265063509461101798 ) ) ;
#60064=LINE ( 'NONE', #99971, #96070 ) ;
#60065=CARTESIAN_POINT ( 'NONE',  ( -5.000000000000022204, 12.50000000000000000, 3.637306695894644726 ) ) ;
#60066=DIRECTION ( 'NONE',  ( -0.000000000000000000, -1.000000000000000000, -0.000000000000000000 ) ) ;
#60067=CIRCLE ( 'NONE', #62213, 0.06509327318403743123 ) ;
#60068=DIRECTION ( 'NONE',  ( -0.000000000000000000, 1.000000000000000000, -0.000000000000000000 ) ) ;
#60069=DIRECTION ( 'NONE',  ( 0.000000000000000000, -0.9999939076577903929, 0.003490651415223739937 ) ) ;
#60070=EDGE_LOOP ( 'NONE', ( #75283, #118676 ) ) ;
#60071=EDGE_LOOP ( 'NONE', ( #26465, #102924, #92245, #33980 ) ) ;
#60072=EDGE_LOOP ( 'NONE', ( #10177, #32505, #52450, #10306 ) ) ;
#60073=ORIENTED_EDGE ( 'NONE', *, *, #76093, .F. ) ;
#60074=CARTESIAN_POINT ( 'NONE',  ( -5.650000000000023448, 2.500000000000000000, -6.841600689897078702 ) ) ;
#60075=DIRECTION ( 'NONE',  ( -4.274815082592931898E-19, -0.9999939076577903929, -0.003490651415223739937 ) ) ;
#60076=FACE_BOUND ( 'NONE', #79707, .T. ) ;
#60077=DIRECTION ( 'NONE',  ( -0.000000000000000000, -1.000000000000000000, -0.000000000000000000 ) ) ;
#60078=AXIS2_PLACEMENT_3D ( 'NONE', #120943, #101319, #31933 ) ;
#60079=CONICAL_SURFACE ( 'NONE', #32983, 0.1000000000000000472, 0.003490658503988666988 ) ;
#60080=EDGE_LOOP ( 'NONE', ( #4194, #32685, #70701, #88727 ) ) ;
#60081=DIRECTION ( 'NONE',  ( 0.000000000000000000, 0.000000000000000000, 1.000000000000000000 ) ) ;
#60082=CARTESIAN_POINT ( 'NONE',  ( 105.5000000000000142, -1.500000000000000222, -1.322875655532295136 ) ) ;
#60083=CARTESIAN_POINT ( 'NONE',  ( 12.29999999999990301, 2.500000000000000000, -0.2464101615137782308 ) ) ;
#60084=CARTESIAN_POINT ( 'NONE',  ( 8.349999999999923261, 2.500000000000000000, -7.188010851410854052 ) ) ;
#60085=ORIENTED_EDGE ( 'NONE', *, *, #80658, .F. ) ;
#60086=DIRECTION ( 'NONE',  ( 0.000000000000000000, 0.000000000000000000, -1.000000000000000000 ) ) ;
#60087=AXIS2_PLACEMENT_3D ( 'NONE', #48402, #18924, #79171 ) ;
#60088=EDGE_CURVE ( 'NONE', #7453, #61323, #1059, .T. ) ;
#60089=VECTOR ( 'NONE', #64284, 1000.000000000000000 ) ;
#60090=ORIENTED_EDGE ( 'NONE', *, *, #50891, .F. ) ;
#60091=VERTEX_POINT ( 'NONE', #18177 ) ;
#60092=EDGE_CURVE ( 'NONE', #98931, #36138, #90125, .T. ) ;
#60093=DIRECTION ( 'NONE',  ( 0.000000000000000000, 0.000000000000000000, -1.000000000000000000 ) ) ;
#60094=DIRECTION ( 'NONE',  ( 0.000000000000000000, -0.000000000000000000, 1.000000000000000000 ) ) ;
#60095=ADVANCED_FACE ( 'NONE', ( #19466 ), #15620, .T. ) ;
#60096=VERTEX_POINT ( 'NONE', #108492 ) ;
#60097=VECTOR ( 'NONE', #15377, 1000.000000000000000 ) ;
#60098=AXIS2_PLACEMENT_3D ( 'NONE', #75178, #35269, #124285 ) ;
#60099=EDGE_CURVE ( 'NONE', #122658, #98888, #17779, .T. ) ;
#60100=VECTOR ( 'NONE', #94345, 1000.000000000000000 ) ;
#60101=CARTESIAN_POINT ( 'NONE',  ( -7.500000000000016875, 12.50000000000000000, -3.637306695894650055 ) ) ;
#60102=DIRECTION ( 'NONE',  ( 0.000000000000000000, -0.000000000000000000, 1.000000000000000000 ) ) ;
#60103=FACE_OUTER_BOUND ( 'NONE', #30484, .T. ) ;
#60104=EDGE_CURVE ( 'NONE', #53570, #1964, #98663, .T. ) ;
#60105=ORIENTED_EDGE ( 'NONE', *, *, #115605, .F. ) ;
#60106=FACE_OUTER_BOUND ( 'NONE', #274, .T. ) ;
#60107=ORIENTED_EDGE ( 'NONE', *, *, #23526, .F. ) ;
#60108=CARTESIAN_POINT ( 'NONE',  ( 12.04999999999990479, 2.500000000000000000, -6.395190528383301931 ) ) ;
#60109=EDGE_CURVE ( 'NONE', #36539, #72573, #13573, .T. ) ;
#60110=ADVANCED_FACE ( 'NONE', ( #72448 ), #111798, .T. ) ;
#60111=ORIENTED_EDGE ( 'NONE', *, *, #27070, .F. ) ;
#60113=VERTEX_POINT ( 'NONE', #52161 ) ;
#60114=DIRECTION ( 'NONE',  ( 0.000000000000000000, 0.000000000000000000, 1.000000000000000000 ) ) ;
#60115=AXIS2_PLACEMENT_3D ( 'NONE', #32584, #81649, #22757 ) ;
#60116=PLANE ( 'NONE',  #121946 ) ;
#60117=PLANE ( 'NONE',  #119852 ) ;
#60118=CARTESIAN_POINT ( 'NONE',  ( -4.999999999999990230, 2.500000000000000000, -4.230127018922201998 ) ) ;
#60119=DIRECTION ( 'NONE',  ( -0.000000000000000000, -1.000000000000000000, -0.000000000000000000 ) ) ;
#60120=AXIS2_PLACEMENT_3D ( 'NONE', #29357, #39826, #119641 ) ;
#60121=ORIENTED_EDGE ( 'NONE', *, *, #48469, .T. ) ;
#60122=CIRCLE ( 'NONE', #22471, 0.06509327318403745899 ) ;
#60123=ORIENTED_EDGE ( 'NONE', *, *, #26019, .T. ) ;
#60124=ORIENTED_EDGE ( 'NONE', *, *, #28186, .F. ) ;
#60125=CARTESIAN_POINT ( 'NONE',  ( 1.249999999999988898, 12.50000000000000000, -6.560283801567339701 ) ) ;
#60126=AXIS2_PLACEMENT_3D ( 'NONE', #81432, #22525, #23142 ) ;
#60127=CARTESIAN_POINT ( 'NONE',  ( 9.349999999999919709, 2.500000000000000000, 1.818653347947321475 ) ) ;
#60128=LINE ( 'NONE', #70562, #110724 ) ;
#60129=ORIENTED_EDGE ( 'NONE', *, *, #101603, .T. ) ;
#60130=ORIENTED_EDGE ( 'NONE', *, *, #111932, .F. ) ;
#60131=VERTEX_POINT ( 'NONE', #12847 ) ;
#60132=CARTESIAN_POINT ( 'NONE',  ( -9.350000000000004974, 2.500000000000000000, 6.941600689897073018 ) ) ;
#60133=CIRCLE ( 'NONE', #35001, 0.06509327318403745899 ) ;
#60134=CONICAL_SURFACE ( 'NONE', #53854, 0.1000000000000002554, 0.003490658503988666988 ) ;
#60135=ORIENTED_EDGE ( 'NONE', *, *, #50162, .F. ) ;
#60136=CARTESIAN_POINT ( 'NONE',  ( 9.149999999999915090, 2.500000000000000000, 6.495190528383297135 ) ) ;
#60137=AXIS2_PLACEMENT_3D ( 'NONE', #125639, #16318, #114531 ) ;
#60138=CONICAL_SURFACE ( 'NONE', #39214, 0.09999999999999982514, 0.003490658503988666988 ) ;
#60139=CARTESIAN_POINT ( 'NONE',  ( -10.45000000000000462, 2.500000000000000000, -6.495190528383298911 ) ) ;
#60140=CARTESIAN_POINT ( 'NONE',  ( -8.750000000000010658, 12.50000000000000000, -1.407149913249512663 ) ) ;
#60141=CARTESIAN_POINT ( 'NONE',  ( -1.900000000000034106, 2.500000000000000000, -3.883716857408426648 ) ) ;
#60142=DIRECTION ( 'NONE',  ( 0.000000000000000000, 0.000000000000000000, -1.000000000000000000 ) ) ;
#60144=VECTOR ( 'NONE', #17583, 1000.000000000000000 ) ;
#60145=DIRECTION ( 'NONE',  ( 0.000000000000000000, -0.000000000000000000, 1.000000000000000000 ) ) ;
#60146=EDGE_LOOP ( 'NONE', ( #40471, #89006, #7961, #85291 ) ) ;
#60148=DIRECTION ( 'NONE',  ( 0.000000000000000000, 0.000000000000000000, 1.000000000000000000 ) ) ;
#60149=AXIS2_PLACEMENT_3D ( 'NONE', #80219, #128019, #107735 ) ;
#60150=VERTEX_POINT ( 'NONE', #101905 ) ;
#60152=VERTEX_POINT ( 'NONE', #122197 ) ;
#60154=DIRECTION ( 'NONE',  ( -0.000000000000000000, 1.000000000000000000, -0.000000000000000000 ) ) ;
#60155=DIRECTION ( 'NONE',  ( 0.000000000000000000, 1.000000000000000000, 0.000000000000000000 ) ) ;
#60156=DIRECTION ( 'NONE',  ( 0.000000000000000000, 1.000000000000000000, 0.000000000000000000 ) ) ;
#60157=ADVANCED_FACE ( 'NONE', ( #1753 ), #12218, .T. ) ;
#60158=CARTESIAN_POINT ( 'NONE',  ( 10.64999999999991331, 2.500000000000000000, -1.818653347947325916 ) ) ;
#60159=DIRECTION ( 'NONE',  ( -0.000000000000000000, -1.000000000000000000, -0.000000000000000000 ) ) ;
#60160=DIRECTION ( 'NONE',  ( -0.000000000000000000, -1.000000000000000000, -0.000000000000000000 ) ) ;
#60161=CIRCLE ( 'NONE', #99860, 0.06509327318403745899 ) ;
#60162=CARTESIAN_POINT ( 'NONE',  ( 10.64999999999991331, 12.50000000000000000, 6.083687093685483660 ) ) ;
#60163=ORIENTED_EDGE ( 'NONE', *, *, #126420, .F. ) ;
#60164=VERTEX_POINT ( 'NONE', #21401 ) ;
#60165=ORIENTED_EDGE ( 'NONE', *, *, #51232, .T. ) ;
#60166=ORIENTED_EDGE ( 'NONE', *, *, #111947, .T. ) ;
#60167=CARTESIAN_POINT ( 'NONE',  ( -4.150000000000027889, 12.50000000000000000, -6.430097255199264339 ) ) ;
#60168=DIRECTION ( 'NONE',  ( -0.000000000000000000, -1.000000000000000000, -0.000000000000000000 ) ) ;
#60169=EDGE_LOOP ( 'NONE', ( #96013, #1718, #35478, #115034 ) ) ;
#60170=AXIS2_PLACEMENT_3D ( 'NONE', #98402, #69597, #80070 ) ;
#60171=LINE ( 'NONE', #119707, #109225 ) ;
#60172=AXIS2_PLACEMENT_3D ( 'NONE', #98308, #7998, #89789 ) ;
#60173=CARTESIAN_POINT ( 'NONE',  ( 4.999999999999935163, 2.500000000000000000, 3.537306695894645081 ) ) ;
#60174=DIRECTION ( 'NONE',  ( -4.274815082592931898E-19, -0.9999939076577903929, -0.003490651415223739937 ) ) ;
#60175=CARTESIAN_POINT ( 'NONE',  ( -9.600000000000008527, 12.50000000000000000, 4.330127018922196314 ) ) ;
#60176=VERTEX_POINT ( 'NONE', #61337 ) ;
#60177=CARTESIAN_POINT ( 'NONE',  ( -9.350000000000004974, 2.500000000000000000, 6.248780366869521430 ) ) ;
#60178=AXIS2_PLACEMENT_3D ( 'NONE', #47411, #76866, #87311 ) ;
#60179=CARTESIAN_POINT ( 'NONE',  ( 11.89999999999990798, 2.500000000000000000, 4.083716857408421497 ) ) ;
#60180=ORIENTED_EDGE ( 'NONE', *, *, #39381, .F. ) ;
#60181=CONICAL_SURFACE ( 'NONE', #93612, 0.09999999999999982514, 0.003490658503988666988 ) ;
#60182=VECTOR ( 'NONE', #128539, 1000.000000000000000 ) ;
#60183=VERTEX_POINT ( 'NONE', #92732 ) ;
#60184=ORIENTED_EDGE ( 'NONE', *, *, #5771, .T. ) ;
#60185=VERTEX_POINT ( 'NONE', #73714 ) ;
#60186=FACE_OUTER_BOUND ( 'NONE', #12896, .T. ) ;
#60187=CARTESIAN_POINT ( 'NONE',  ( -4.999999999999986677, 2.500000000000000000, 4.330127018922196314 ) ) ;
#60188=DIRECTION ( 'NONE',  ( -0.000000000000000000, 1.000000000000000000, -0.000000000000000000 ) ) ;
#60189=AXIS2_PLACEMENT_3D ( 'NONE', #17710, #37382, #26268 ) ;
#60190=EDGE_CURVE ( 'NONE', #58954, #89885, #113654, .T. ) ;
#60191=DIRECTION ( 'NONE',  ( 0.000000000000000000, 0.000000000000000000, 1.000000000000000000 ) ) ;
#60192=VERTEX_POINT ( 'NONE', #63915 ) ;
#60193=AXIS2_PLACEMENT_3D ( 'NONE', #32324, #110216, #241 ) ;
#60194=DIRECTION ( 'NONE',  ( -0.000000000000000000, -1.000000000000000000, -0.000000000000000000 ) ) ;
#60195=CARTESIAN_POINT ( 'NONE',  ( 11.24999999999994316, 12.50000000000000000, -6.560283801567339701 ) ) ;
#60196=ADVANCED_FACE ( 'NONE', ( #92067 ), #49110, .T. ) ;
#60197=DIRECTION ( 'NONE',  ( 0.000000000000000000, 1.000000000000000000, 0.000000000000000000 ) ) ;
#60198=CARTESIAN_POINT ( 'NONE',  ( 10.84999999999990905, 12.50000000000000000, 1.472243186433545459 ) ) ;
#60199=EDGE_CURVE ( 'NONE', #9486, #70431, #122267, .T. ) ;
#60200=ORIENTED_EDGE ( 'NONE', *, *, #49690, .T. ) ;
#60201=CONICAL_SURFACE ( 'NONE', #97826, 0.1000000000000002554, 0.003490658503988666988 ) ;
#60202=CARTESIAN_POINT ( 'NONE',  ( 11.24999999999990585, 2.500000000000000000, 2.957883832488649389 ) ) ;
#60203=AXIS2_PLACEMENT_3D ( 'NONE', #87290, #89873, #127867 ) ;
#60204=EDGE_LOOP ( 'NONE', ( #84841, #34140, #48171, #10157 ) ) ;
#60206=ADVANCED_FACE ( 'NONE', ( #3066 ), #9391, .T. ) ;
#60207=ORIENTED_EDGE ( 'NONE', *, *, #52414, .F. ) ;
#60208=DIRECTION ( 'NONE',  ( 0.000000000000000000, 0.000000000000000000, -1.000000000000000000 ) ) ;
#60209=ADVANCED_FACE ( 'NONE', ( #22071 ), #84683, .T. ) ;
#60210=DIRECTION ( 'NONE',  ( 0.000000000000000000, 0.000000000000000000, -1.000000000000000000 ) ) ;
#60211=EDGE_CURVE ( 'NONE', #6145, #46603, #11526, .T. ) ;
#60212=FACE_BOUND ( 'NONE', #57934, .T. ) ;
#60213=VECTOR ( 'NONE', #59149, 1000.000000000000000 ) ;
#60215=DIRECTION ( 'NONE',  ( 0.000000000000000000, 1.000000000000000000, 0.000000000000000000 ) ) ;
#60216=VECTOR ( 'NONE', #8562, 1000.000000000000000 ) ;
#60217=CARTESIAN_POINT ( 'NONE',  ( 6.249999999999928946, 2.500000000000000000, 2.857883832488649301 ) ) ;
#60218=CONICAL_SURFACE ( 'NONE', #47682, 0.09999999999999982514, 0.003490658503988666988 ) ;
#60219=DIRECTION ( 'NONE',  ( 0.000000000000000000, -0.000000000000000000, 1.000000000000000000 ) ) ;
#60220=DIRECTION ( 'NONE',  ( 0.000000000000000000, -0.000000000000000000, 1.000000000000000000 ) ) ;
#60221=EDGE_CURVE ( 'NONE', #13533, #35640, #102537, .T. ) ;
#60222=CIRCLE ( 'NONE', #72722, 0.06509327318403745899 ) ;
#60223=DIRECTION ( 'NONE',  ( 0.000000000000000000, 0.000000000000000000, -1.000000000000000000 ) ) ;
#60224=AXIS2_PLACEMENT_3D ( 'NONE', #4192, #74248, #124637 ) ;
#60225=CARTESIAN_POINT ( 'NONE',  ( 9.599999999999917932, 2.500000000000000000, 0.6928203230275494784 ) ) ;
#60226=ORIENTED_EDGE ( 'NONE', *, *, #108514, .F. ) ;
#60227=FACE_OUTER_BOUND ( 'NONE', #3700, .T. ) ;
#60228=VECTOR ( 'NONE', #101074, 1000.000000000000000 ) ;
#60230=ORIENTED_EDGE ( 'NONE', *, *, #38758, .T. ) ;
#60231=EDGE_LOOP ( 'NONE', ( #118855, #117963, #87621, #112125 ) ) ;
#60232=DIRECTION ( 'NONE',  ( -0.000000000000000000, 1.000000000000000000, -0.000000000000000000 ) ) ;
#60233=VECTOR ( 'NONE', #23383, 1000.000000000000000 ) ;
#60234=CARTESIAN_POINT ( 'NONE',  ( -14.14999999999998614, 2.500000000000000000, -2.065063509461099844 ) ) ;
#60235=FACE_BOUND ( 'NONE', #32748, .T. ) ;
#60236=DIRECTION ( 'NONE',  ( 0.000000000000000000, 1.000000000000000000, 0.000000000000000000 ) ) ;
#60237=CIRCLE ( 'NONE', #76938, 0.06509327318403745899 ) ;
#60238=CIRCLE ( 'NONE', #85345, 0.06509327318403745899 ) ;
#60239=CARTESIAN_POINT ( 'NONE',  ( -2.500000000000032863, 2.500000000000000000, 5.122947341949749323 ) ) ;
#60240=EDGE_LOOP ( 'NONE', ( #60090, #128234, #88438, #50362 ) ) ;
#60241=DIRECTION ( 'NONE',  ( -0.000000000000000000, -1.000000000000000000, -0.000000000000000000 ) ) ;
#60242=EDGE_CURVE ( 'NONE', #77368, #87565, #95256, .T. ) ;
#60244=ORIENTED_EDGE ( 'NONE', *, *, #123171, .T. ) ;
#60245=DIRECTION ( 'NONE',  ( 0.000000000000000000, 0.000000000000000000, 1.000000000000000000 ) ) ;
#60246=CARTESIAN_POINT ( 'NONE',  ( 2.949999999999943334, 2.500000000000000000, 6.495190528383297135 ) ) ;
#60248=EDGE_CURVE ( 'NONE', #2963, #84112, #84781, .T. ) ;
#60249=CARTESIAN_POINT ( 'NONE',  ( -14.19999999999998685, 2.500000000000000000, -1.084202172485504434E-16 ) ) ;
#60251=EDGE_CURVE ( 'NONE', #116584, #105882, #71804, .T. ) ;
#60253=EDGE_CURVE ( 'NONE', #125089, #63009, #53457, .T. ) ;
#60254=DIRECTION ( 'NONE',  ( -0.000000000000000000, 1.000000000000000000, -0.000000000000000000 ) ) ;
#60255=AXIS2_PLACEMENT_3D ( 'NONE', #11127, #31442, #120455 ) ;
#60256=DIRECTION ( 'NONE',  ( 0.000000000000000000, 0.000000000000000000, 1.000000000000000000 ) ) ;
#60257=DIRECTION ( 'NONE',  ( -0.000000000000000000, 1.000000000000000000, -0.000000000000000000 ) ) ;
#60258=EDGE_CURVE ( 'NONE', #92344, #101832, #19946, .T. ) ;
#60260=AXIS2_PLACEMENT_3D ( 'NONE', #31909, #71837, #62018 ) ;
#60261=ORIENTED_EDGE ( 'NONE', *, *, #20947, .F. ) ;
#60262=ADVANCED_FACE ( 'NONE', ( #55382 ), #55446, .T. ) ;
#60263=DIRECTION ( 'NONE',  ( 0.000000000000000000, 0.000000000000000000, -1.000000000000000000 ) ) ;
#60264=EDGE_CURVE ( 'NONE', #6155, #55060, #76954, .T. ) ;
#60265=VERTEX_POINT ( 'NONE', #105108 ) ;
#60266=DIRECTION ( 'NONE',  ( -0.000000000000000000, -1.000000000000000000, -0.000000000000000000 ) ) ;
#60267=CARTESIAN_POINT ( 'NONE',  ( 17.50000000000000000, -2.499999999999999556, -2.333333333333329040 ) ) ;
#60268=CIRCLE ( 'NONE', #53893, 0.1000000000000002554 ) ;
#60269=EDGE_CURVE ( 'NONE', #63941, #98238, #126553, .T. ) ;
#60270=AXIS2_PLACEMENT_3D ( 'NONE', #33249, #51596, #23393 ) ;
#60271=EDGE_CURVE ( 'NONE', #99984, #54010, #66476, .T. ) ;
#60273=ORIENTED_EDGE ( 'NONE', *, *, #52068, .F. ) ;
#60274=CARTESIAN_POINT ( 'NONE',  ( 7.099999999999928590, 12.50000000000000000, 4.265033745738159077 ) ) ;
#60275=DIRECTION ( 'NONE',  ( 0.000000000000000000, -0.000000000000000000, 1.000000000000000000 ) ) ;
#60276=DIRECTION ( 'NONE',  ( 0.000000000000000000, 0.000000000000000000, -1.000000000000000000 ) ) ;
#60277=DIRECTION ( 'NONE',  ( 0.000000000000000000, 0.000000000000000000, 1.000000000000000000 ) ) ;
#60278=LINE ( 'NONE', #119167, #19398 ) ;
#60279=CARTESIAN_POINT ( 'NONE',  ( -10.65000000000000213, 12.50000000000000000, 6.841600689897072485 ) ) ;
#60280=EDGE_CURVE ( 'NONE', #21509, #91809, #107766, .T. ) ;
#60281=CONICAL_SURFACE ( 'NONE', #79144, 0.1000000000000002554, 0.003490658503988666988 ) ;
#60282=ORIENTED_EDGE ( 'NONE', *, *, #47485, .F. ) ;
#60283=AXIS2_PLACEMENT_3D ( 'NONE', #83802, #72072, #41329 ) ;
#60284=EDGE_LOOP ( 'NONE', ( #13103, #96356 ) ) ;
#60285=CARTESIAN_POINT ( 'NONE',  ( -1.250000000000036193, 12.50000000000000000, 5.802370205355744659 ) ) ;
#60286=ORIENTED_EDGE ( 'NONE', *, *, #60627, .T. ) ;
#60287=CARTESIAN_POINT ( 'NONE',  ( 7.099999999999928590, 2.500000000000000000, -4.330127018922201643 ) ) ;
#60288=VERTEX_POINT ( 'NONE', #96571 ) ;
#60290=VERTEX_POINT ( 'NONE', #76313 ) ;
#60291=CARTESIAN_POINT ( 'NONE',  ( 87.50000000000001421, -3.974992050023848922, -6.359987280038160051 ) ) ;
#60292=VECTOR ( 'NONE', #13693, 1000.000000000000000 ) ;
#60293=DIRECTION ( 'NONE',  ( 0.000000000000000000, -0.000000000000000000, 1.000000000000000000 ) ) ;
#60294=FACE_OUTER_BOUND ( 'NONE', #107726, .T. ) ;
#60296=FACE_OUTER_BOUND ( 'NONE', #103250, .T. ) ;
#60297=DIRECTION ( 'NONE',  ( 0.000000000000000000, 0.000000000000000000, -1.000000000000000000 ) ) ;
#60298=CARTESIAN_POINT ( 'NONE',  ( 1.899999999999949507, 2.500000000000000000, 4.676537180435972552 ) ) ;
#60299=CARTESIAN_POINT ( 'NONE',  ( 6.049999999999934097, 2.500000000000000000, -6.148780366869526226 ) ) ;
#60300=DIRECTION ( 'NONE',  ( 0.000000000000000000, 0.000000000000000000, 1.000000000000000000 ) ) ;
#60301=DIRECTION ( 'NONE',  ( -4.274815082592931898E-19, -0.9999939076577903929, -0.003490651415223739937 ) ) ;
#60302=AXIS2_PLACEMENT_3D ( 'NONE', #73181, #5709, #84280 ) ;
#60303=EDGE_LOOP ( 'NONE', ( #32272, #69078, #88732, #108318 ) ) ;
#60305=ORIENTED_EDGE ( 'NONE', *, *, #27082, .F. ) ;
#60306=ORIENTED_EDGE ( 'NONE', *, *, #119902, .F. ) ;
#60307=CARTESIAN_POINT ( 'NONE',  ( -10.40000000000000213, 12.50000000000000000, 4.957854068765711553 ) ) ;
#60308=AXIS2_PLACEMENT_3D ( 'NONE', #34028, #45151, #73954 ) ;
#60309=DIRECTION ( 'NONE',  ( -0.000000000000000000, -1.000000000000000000, -0.000000000000000000 ) ) ;
#60311=CONICAL_SURFACE ( 'NONE', #97934, 0.1000000000000000472, 0.003490658503988666988 ) ;
#60312=EDGE_CURVE ( 'NONE', #13780, #74146, #80587, .T. ) ;
#60313=DIRECTION ( 'NONE',  ( 0.000000000000000000, 0.000000000000000000, 1.000000000000000000 ) ) ;
#60314=DIRECTION ( 'NONE',  ( 0.000000000000000000, 0.000000000000000000, 1.000000000000000000 ) ) ;
#60315=CARTESIAN_POINT ( 'NONE',  ( 1.249999999999988454, 2.500000000000000000, 2.265063509461097357 ) ) ;
#60316=EDGE_LOOP ( 'NONE', ( #30248, #102633, #26575, #42575 ) ) ;
#60317=AXIS2_PLACEMENT_3D ( 'NONE', #77298, #64889, #117188 ) ;
#60318=VERTEX_POINT ( 'NONE', #105770 ) ;
#60319=CARTESIAN_POINT ( 'NONE',  ( -4.150000000000025224, 2.500000000000000000, -1.472243186433550122 ) ) ;
#60320=ORIENTED_EDGE ( 'NONE', *, *, #112518, .T. ) ;
#60321=CARTESIAN_POINT ( 'NONE',  ( -7.950000000000009059, 2.500000000000000000, 6.595190528383296780 ) ) ;
#60322=ORIENTED_EDGE ( 'NONE', *, *, #4794, .F. ) ;
#60323=AXIS2_PLACEMENT_3D ( 'NONE', #63602, #11908, #72133 ) ;
#60324=ADVANCED_FACE ( 'NONE', ( #4970 ), #72189, .T. ) ;
#60325=ORIENTED_EDGE ( 'NONE', *, *, #26819, .T. ) ;
#60326=CARTESIAN_POINT ( 'NONE',  ( 2.899999999999946620, 2.500000000000000000, 0.6928203230275494784 ) ) ;
#60327=CARTESIAN_POINT ( 'NONE',  ( 26.74601813931272787, -2.978655629156510276, -2.722801754518478390 ) ) ;
#60328=CARTESIAN_POINT ( 'NONE',  ( 9.149999999999918643, 2.500000000000000000, -6.495190528383302464 ) ) ;
#60329=FACE_OUTER_BOUND ( 'NONE', #123297, .T. ) ;
#60330=CARTESIAN_POINT ( 'NONE',  ( 87.50000000000002842, 2.781865847474099152, 7.000342182495696619 ) ) ;
#60331=VERTEX_POINT ( 'NONE', #116860 ) ;
#60332=DIRECTION ( 'NONE',  ( -4.274815082592931898E-19, -0.9999939076577903929, -0.003490651415223739937 ) ) ;
#60333=DIRECTION ( 'NONE',  ( -0.000000000000000000, 1.000000000000000000, -0.000000000000000000 ) ) ;
#60334=FACE_OUTER_BOUND ( 'NONE', #88762, .T. ) ;
#60335=CARTESIAN_POINT ( 'NONE',  ( -12.04999999999999716, 12.50000000000000000, -6.495190528383298911 ) ) ;
#60336=DIRECTION ( 'NONE',  ( 0.000000000000000000, 1.000000000000000000, 0.000000000000000000 ) ) ;
#60337=VERTEX_POINT ( 'NONE', #6891 ) ;
#60338=ORIENTED_EDGE ( 'NONE', *, *, #106059, .F. ) ;
#60339=AXIS2_PLACEMENT_3D ( 'NONE', #119779, #11757, #121072 ) ;
#60340=CARTESIAN_POINT ( 'NONE',  ( -8.749999999999971578, 2.500000000000000000, 6.495190528383297135 ) ) ;
#60341=ORIENTED_EDGE ( 'NONE', *, *, #100274, .T. ) ;
#60342=CARTESIAN_POINT ( 'NONE',  ( -11.44999999999999751, 2.500000000000000000, 6.148780366869520897 ) ) ;
#60343=CARTESIAN_POINT ( 'NONE',  ( -6.650000000000018119, 2.500000000000000000, -2.757883832488654097 ) ) ;
#60344=CIRCLE ( 'NONE', #118809, 0.06509327318403745899 ) ;
#60345=ADVANCED_FACE ( 'NONE', ( #74373 ), #7396, .T. ) ;
#60346=CIRCLE ( 'NONE', #102192, 0.06509327318403745899 ) ;
#60347=CIRCLE ( 'NONE', #3882, 0.09999999999999982514 ) ;
#60348=VERTEX_POINT ( 'NONE', #5609 ) ;
#60349=CARTESIAN_POINT ( 'NONE',  ( -11.05000000000000071, 12.50000000000000000, 2.511473670974873507 ) ) ;
#60350=CARTESIAN_POINT ( 'NONE',  ( -10.40000000000000213, 2.500000000000000000, -2.276824562219559311E-15 ) ) ;
#60351=DIRECTION ( 'NONE',  ( -0.000000000000000000, -1.000000000000000000, -0.000000000000000000 ) ) ;
#60352=DIRECTION ( 'NONE',  ( 0.000000000000000000, 0.000000000000000000, 1.000000000000000000 ) ) ;
#60353=ADVANCED_FACE ( 'NONE', ( #25924 ), #16712, .T. ) ;
#60354=VECTOR ( 'NONE', #7595, 1000.000000000000000 ) ;
#60355=AXIS2_PLACEMENT_3D ( 'NONE', #43233, #3924, #74604 ) ;
#60356=CIRCLE ( 'NONE', #93795, 0.09999999999999999167 ) ;
#60357=DIRECTION ( 'NONE',  ( 0.000000000000000000, 0.000000000000000000, 1.000000000000000000 ) ) ;
#60358=CIRCLE ( 'NONE', #20639, 0.06509327318403745899 ) ;
#60359=ORIENTED_EDGE ( 'NONE', *, *, #75707, .T. ) ;
#60360=ADVANCED_FACE ( 'NONE', ( #106405 ), #86761, .T. ) ;
#60361=ADVANCED_FACE ( 'NONE', ( #94010 ), #15717, .T. ) ;
#60362=EDGE_CURVE ( 'NONE', #11624, #14537, #32489, .T. ) ;
#60363=CARTESIAN_POINT ( 'NONE',  ( 43.31231356391106857, 3.511368398499961963, -3.941707252993503552 ) ) ;
#60364=EDGE_CURVE ( 'NONE', #85762, #46426, #88895, .T. ) ;
#60365=EDGE_CURVE ( 'NONE', #29752, #30275, #76383, .T. ) ;
#60366=LINE ( 'NONE', #30900, #83307 ) ;
#60367=VECTOR ( 'NONE', #8822, 1000.000000000000000 ) ;
#60368=DIRECTION ( 'NONE',  ( 0.000000000000000000, -0.000000000000000000, 1.000000000000000000 ) ) ;
#60369=CARTESIAN_POINT ( 'NONE',  ( -12.49999999999999289, 2.500000000000000000, -0.5928203230275499447 ) ) ;
#60370=AXIS2_PLACEMENT_3D ( 'NONE', #115170, #109233, #98775 ) ;
#60371=EDGE_LOOP ( 'NONE', ( #24049, #2131, #77614, #98881 ) ) ;
#60372=ORIENTED_EDGE ( 'NONE', *, *, #87527, .F. ) ;
#60373=FACE_OUTER_BOUND ( 'NONE', #84208, .T. ) ;
#60374=DIRECTION ( 'NONE',  ( 0.000000000000000000, 1.000000000000000000, 0.000000000000000000 ) ) ;
#60375=ADVANCED_FACE ( 'NONE', ( #94644 ), #124507, .T. ) ;
#60376=DIRECTION ( 'NONE',  ( 0.000000000000000000, 1.000000000000000000, 0.000000000000000000 ) ) ;
#60377=ORIENTED_EDGE ( 'NONE', *, *, #122981, .T. ) ;
#60378=ADVANCED_FACE ( 'NONE', ( #116218 ), #107041, .T. ) ;
#60379=PLANE ( 'NONE',  #128376 ) ;
#60380=EDGE_CURVE ( 'NONE', #114224, #113778, #97873, .T. ) ;
#60381=DIRECTION ( 'NONE',  ( -0.000000000000000000, 1.000000000000000000, -0.000000000000000000 ) ) ;
#60382=AXIS2_PLACEMENT_3D ( 'NONE', #119228, #36817, #29559 ) ;
#60383=VERTEX_POINT ( 'NONE', #10149 ) ;
#60384=CARTESIAN_POINT ( 'NONE',  ( 5.849999999999932143, 12.50000000000000000, 1.537336459617582918 ) ) ;
#60385=VERTEX_POINT ( 'NONE', #99827 ) ;
#60386=CARTESIAN_POINT ( 'NONE',  ( 13.09999999999990195, 2.500000000000000000, -3.983716857408426293 ) ) ;
#60387=ORIENTED_EDGE ( 'NONE', *, *, #129498, .F. ) ;
#60388=VECTOR ( 'NONE', #26504, 1000.000000000000000 ) ;
#60389=CARTESIAN_POINT ( 'NONE',  ( 2.049999999999948308, 12.50000000000000000, 6.430097255199259010 ) ) ;
#60390=DIRECTION ( 'NONE',  ( 0.000000000000000000, 0.000000000000000000, -1.000000000000000000 ) ) ;
#60391=ORIENTED_EDGE ( 'NONE', *, *, #66047, .T. ) ;
#60392=ORIENTED_EDGE ( 'NONE', *, *, #48595, .T. ) ;
#60393=CARTESIAN_POINT ( 'NONE',  ( 9.149999999999920419, 2.500000000000000000, 2.757883832488649656 ) ) ;
#60395=CIRCLE ( 'NONE', #91476, 0.06509327318403745899 ) ;
#60396=VERTEX_POINT ( 'NONE', #127986 ) ;
#60397=DIRECTION ( 'NONE',  ( 0.000000000000000000, -0.000000000000000000, 1.000000000000000000 ) ) ;
#60399=AXIS2_PLACEMENT_3D ( 'NONE', #112662, #64834, #55015 ) ;
#60400=FACE_OUTER_BOUND ( 'NONE', #21974, .T. ) ;
#60402=CARTESIAN_POINT ( 'NONE',  ( 7.099999999999925926, 2.500000000000000000, 0.6928203230275494784 ) ) ;
#60403=CARTESIAN_POINT ( 'NONE',  ( 4.799999999999937650, 2.500000000000000000, -0.2464101615137782308 ) ) ;
#60404=DIRECTION ( 'NONE',  ( 0.000000000000000000, 1.000000000000000000, 0.000000000000000000 ) ) ;
#60405=ORIENTED_EDGE ( 'NONE', *, *, #55756, .T. ) ;
#60406=EDGE_LOOP ( 'NONE', ( #65729, #42670, #99590, #84511 ) ) ;
#60407=CIRCLE ( 'NONE', #10217, 0.1000000000000000472 ) ;
#60408=VECTOR ( 'NONE', #128141, 1000.000000000000000 ) ;
#60410=LINE ( 'NONE', #90472, #41321 ) ;
#60411=DIRECTION ( 'NONE',  ( -0.000000000000000000, 1.000000000000000000, -0.000000000000000000 ) ) ;
#60412=FACE_OUTER_BOUND ( 'NONE', #58802, .T. ) ;
#60413=CONICAL_SURFACE ( 'NONE', #20690, 0.1000000000000002554, 0.003490658503988666988 ) ;
#60414=ORIENTED_EDGE ( 'NONE', *, *, #111334, .F. ) ;
#60415=ORIENTED_EDGE ( 'NONE', *, *, #64225, .T. ) ;
#60416=FACE_BOUND ( 'NONE', #113104, .T. ) ;
#60417=ORIENTED_EDGE ( 'NONE', *, *, #15607, .F. ) ;
#60418=EDGE_CURVE ( 'NONE', #123363, #73897, #45087, .T. ) ;
#60419=CARTESIAN_POINT ( 'NONE',  ( -8.749999999999971578, 12.50000000000000000, 6.430097255199259010 ) ) ;
#60420=CARTESIAN_POINT ( 'NONE',  ( 7.299999999999927880, 2.500000000000000000, -4.776537180435977525 ) ) ;
#60421=ADVANCED_FACE ( 'NONE', ( #59269 ), #57603, .T. ) ;
#60422=CARTESIAN_POINT ( 'NONE',  ( 8.349999999999923261, 12.50000000000000000, 2.165063509461097713 ) ) ;
#60423=CIRCLE ( 'NONE', #50053, 0.06509327318403745899 ) ;
#60425=LINE ( 'NONE', #116244, #128835 ) ;
#60426=EDGE_CURVE ( 'NONE', #28650, #64939, #86831, .T. ) ;
#60427=CARTESIAN_POINT ( 'NONE',  ( -12.09999999999999432, 2.500000000000000000, 3.737306695894644371 ) ) ;
#60428=DIRECTION ( 'NONE',  ( -0.000000000000000000, 1.000000000000000000, -0.000000000000000000 ) ) ;
#60429=DIRECTION ( 'NONE',  ( 0.000000000000000000, 0.000000000000000000, 1.000000000000000000 ) ) ;
#60430=DIRECTION ( 'NONE',  ( -4.274815082592931898E-19, -0.9999939076577903929, -0.003490651415223739937 ) ) ;
#60431=CARTESIAN_POINT ( 'NONE',  ( 5.849999999999934808, 2.500000000000000000, -5.802370205355749988 ) ) ;
#60432=ADVANCED_FACE ( 'NONE', ( #80180 ), #38998, .T. ) ;
#60433=EDGE_LOOP ( 'NONE', ( #64819, #71278, #109671, #89109 ) ) ;
#60434=EDGE_LOOP ( 'NONE', ( #20831, #30571 ) ) ;
#60435=VERTEX_POINT ( 'NONE', #50097 ) ;
#60436=ORIENTED_EDGE ( 'NONE', *, *, #9217, .F. ) ;
#60437=DIRECTION ( 'NONE',  ( 0.000000000000000000, 0.000000000000000000, -1.000000000000000000 ) ) ;
#60438=AXIS2_PLACEMENT_3D ( 'NONE', #28029, #46363, #118336 ) ;
#60439=CARTESIAN_POINT ( 'NONE',  ( -1.650000000000034328, 12.50000000000000000, -7.188010851410854052 ) ) ;
#60440=ORIENTED_EDGE ( 'NONE', *, *, #118604, .T. ) ;
#60441=VERTEX_POINT ( 'NONE', #40261 ) ;
#60442=ORIENTED_EDGE ( 'NONE', *, *, #93887, .F. ) ;
#60443=DIRECTION ( 'NONE',  ( -4.274815082592931898E-19, -0.9999939076577903929, -0.003490651415223739937 ) ) ;
#60444=VECTOR ( 'NONE', #116491, 1000.000000000000000 ) ;
#60445=CIRCLE ( 'NONE', #12383, 0.06509327318403745899 ) ;
#60446=FACE_OUTER_BOUND ( 'NONE', #31347, .T. ) ;
#60448=CARTESIAN_POINT ( 'NONE',  ( 7.899999999999924860, 2.500000000000000000, 3.737306695894644371 ) ) ;
#60449=DIRECTION ( 'NONE',  ( 0.000000000000000000, 0.000000000000000000, 1.000000000000000000 ) ) ;
#60450=CARTESIAN_POINT ( 'NONE',  ( -6.700000000000019718, 12.50000000000000000, 0.06509327318403504425 ) ) ;
#60451=CARTESIAN_POINT ( 'NONE',  ( -15.59999999999998010, 12.50000000000000000, 0.3464101615137759604 ) ) ;
#60452=ADVANCED_FACE ( 'NONE', ( #78261 ), #91043, .T. ) ;
#60453=ORIENTED_EDGE ( 'NONE', *, *, #10352, .T. ) ;
#60454=AXIS2_PLACEMENT_3D ( 'NONE', #66416, #57909, #87972 ) ;
#60455=CIRCLE ( 'NONE', #120974, 0.06509327318403741736 ) ;
#60456=DIRECTION ( 'NONE',  ( -0.000000000000000000, -1.000000000000000000, -0.000000000000000000 ) ) ;
#60457=VERTEX_POINT ( 'NONE', #30455 ) ;
#60458=AXIS2_PLACEMENT_3D ( 'NONE', #107428, #17075, #57694 ) ;
#60459=ORIENTED_EDGE ( 'NONE', *, *, #32132, .T. ) ;
#60460=ORIENTED_EDGE ( 'NONE', *, *, #25619, .F. ) ;
#60461=DIRECTION ( 'NONE',  ( 0.000000000000000000, 0.000000000000000000, 1.000000000000000000 ) ) ;
#60462=ORIENTED_EDGE ( 'NONE', *, *, #12258, .T. ) ;
#60463=ORIENTED_EDGE ( 'NONE', *, *, #82880, .F. ) ;
#60464=AXIS2_PLACEMENT_3D ( 'NONE', #28338, #98341, #67592 ) ;
#60466=AXIS2_PLACEMENT_3D ( 'NONE', #73192, #41819, #52267 ) ;
#60467=CARTESIAN_POINT ( 'NONE',  ( -5.850000000000019185, 2.500000000000000000, 6.495190528383297135 ) ) ;
#60468=CARTESIAN_POINT ( 'NONE',  ( 3.749999999999976907, 2.500000000000000000, 2.165063509461097713 ) ) ;
#60469=EDGE_CURVE ( 'NONE', #36953, #32790, #28354, .T. ) ;
#60470=CARTESIAN_POINT ( 'NONE',  ( -11.84999999999999787, 2.500000000000000000, -1.818653347947321919 ) ) ;
#60471=DIRECTION ( 'NONE',  ( 0.000000000000000000, 0.000000000000000000, -1.000000000000000000 ) ) ;
#60472=CARTESIAN_POINT ( 'NONE',  ( 6.849999999999927702, 12.50000000000000000, 2.446380397790835826 ) ) ;
#60473=DIRECTION ( 'NONE',  ( 0.000000000000000000, -0.9999939076577903929, 0.003490651415223739937 ) ) ;
#60475=DIRECTION ( 'NONE',  ( 0.000000000000000000, 0.000000000000000000, -1.000000000000000000 ) ) ;
#60476=EDGE_LOOP ( 'NONE', ( #67539, #58302, #88436, #98507 ) ) ;
#60478=CARTESIAN_POINT ( 'NONE',  ( 0.4499999999999569344, 2.500000000000000000, -2.265063509461101798 ) ) ;
#60479=AXIS2_PLACEMENT_3D ( 'NONE', #66997, #126589, #48035 ) ;
#60480=ORIENTED_EDGE ( 'NONE', *, *, #116798, .F. ) ;
#60481=CARTESIAN_POINT ( 'NONE',  ( -6.650000000000015454, 2.500000000000000000, 2.857883832488649301 ) ) ;
#60482=ADVANCED_FACE ( 'NONE', ( #19972 ), #27848, .T. ) ;
#60483=DIRECTION ( 'NONE',  ( -0.000000000000000000, -1.000000000000000000, -0.000000000000000000 ) ) ;
#60484=ORIENTED_EDGE ( 'NONE', *, *, #62978, .F. ) ;
#60485=DIRECTION ( 'NONE',  ( 0.000000000000000000, 1.000000000000000000, 0.000000000000000000 ) ) ;
#60486=ORIENTED_EDGE ( 'NONE', *, *, #64937, .T. ) ;
#60487=EDGE_LOOP ( 'NONE', ( #55482, #40221, #41544, #79664 ) ) ;
#60488=CARTESIAN_POINT ( 'NONE',  ( 4.149999999999939959, 2.500000000000000000, 1.372243186433545370 ) ) ;
#60489=DIRECTION ( 'NONE',  ( -0.000000000000000000, 1.000000000000000000, -0.000000000000000000 ) ) ;
#60491=LINE ( 'NONE', #83345, #74358 ) ;
#60492=CIRCLE ( 'NONE', #62629, 0.06509327318403745899 ) ;
#60493=AXIS2_PLACEMENT_3D ( 'NONE', #12822, #80488, #70643 ) ;
#60494=DIRECTION ( 'NONE',  ( 0.000000000000000000, 0.000000000000000000, 1.000000000000000000 ) ) ;
#60495=ORIENTED_EDGE ( 'NONE', *, *, #25960, .F. ) ;
#60496=CARTESIAN_POINT ( 'NONE',  ( -11.84999999999999787, 2.500000000000000000, -6.148780366869522673 ) ) ;
#60497=AXIS2_PLACEMENT_3D ( 'NONE', #36927, #29046, #6776 ) ;
#60498=EDGE_LOOP ( 'NONE', ( #44011, #125722, #28242, #80947 ) ) ;
#60499=CARTESIAN_POINT ( 'NONE',  ( -10.60000000000000142, 2.500000000000000000, 3.983716857408420964 ) ) ;
#60500=CARTESIAN_POINT ( 'NONE',  ( 7.499999999999961808, 2.500000000000000000, -4.430127018922202176 ) ) ;
#60501=ADVANCED_FACE ( 'NONE', ( #29160 ), #61811, .T. ) ;
#60502=AXIS2_PLACEMENT_3D ( 'NONE', #66581, #47607, #19408 ) ;
#60504=DIRECTION ( 'NONE',  ( 0.000000000000000000, 1.000000000000000000, 0.000000000000000000 ) ) ;
#60505=LINE ( 'NONE', #100413, #71609 ) ;
#60507=DIRECTION ( 'NONE',  ( 0.000000000000000000, -0.9999939076577903929, 0.003490651415223739937 ) ) ;
#60508=EDGE_LOOP ( 'NONE', ( #8640, #83828 ) ) ;
#60509=EDGE_CURVE ( 'NONE', #41032, #120360, #78545, .T. ) ;
#60510=CIRCLE ( 'NONE', #58360, 0.06509327318403745899 ) ;
#60511=AXIS2_PLACEMENT_3D ( 'NONE', #109765, #19431, #39116 ) ;
#60513=CARTESIAN_POINT ( 'NONE',  ( 0.5999999999999621192, 2.500000000000000000, 0.3464101615137758494 ) ) ;
#60514=PLANE ( 'NONE',  #60126 ) ;
#60515=EDGE_CURVE ( 'NONE', #3042, #96780, #26303, .T. ) ;
#60516=EDGE_CURVE ( 'NONE', #53654, #90160, #57965, .T. ) ;
#60517=ADVANCED_FACE ( 'NONE', ( #8201 ), #48144, .T. ) ;
#60518=EDGE_CURVE ( 'NONE', #55240, #74476, #39638, .T. ) ;
#60519=VERTEX_POINT ( 'NONE', #98504 ) ;
#60520=DIRECTION ( 'NONE',  ( 0.000000000000000000, 0.000000000000000000, 1.000000000000000000 ) ) ;
#60521=ORIENTED_EDGE ( 'NONE', *, *, #23228, .F. ) ;
#60522=EDGE_LOOP ( 'NONE', ( #49646, #53881, #127856, #77986 ) ) ;
#60523=DIRECTION ( 'NONE',  ( 0.000000000000000000, 0.000000000000000000, 1.000000000000000000 ) ) ;
#60524=EDGE_CURVE ( 'NONE', #79739, #74262, #128731, .T. ) ;
#60525=CIRCLE ( 'NONE', #108522, 0.1000000000000000056 ) ;
#60526=EDGE_CURVE ( 'NONE', #76809, #57584, #82745, .T. ) ;
#60527=ORIENTED_EDGE ( 'NONE', *, *, #21332, .T. ) ;
#60528=DIRECTION ( 'NONE',  ( 0.000000000000000000, 1.000000000000000000, 0.000000000000000000 ) ) ;
#60529=DIRECTION ( 'NONE',  ( -0.000000000000000000, 1.000000000000000000, -0.000000000000000000 ) ) ;
#60530=ADVANCED_FACE ( 'NONE', ( #93227 ), #15815, .T. ) ;
#60531=VERTEX_POINT ( 'NONE', #13356 ) ;
#60532=EDGE_CURVE ( 'NONE', #85431, #112209, #93200, .T. ) ;
#60533=AXIS2_PLACEMENT_3D ( 'NONE', #69010, #128618, #79497 ) ;
#60534=FACE_OUTER_BOUND ( 'NONE', #7337, .T. ) ;
#60535=ADVANCED_FACE ( 'NONE', ( #122043 ), #82108, .T. ) ;
#60536=AXIS2_PLACEMENT_3D ( 'NONE', #36500, #17463, #56728 ) ;
#60537=CARTESIAN_POINT ( 'NONE',  ( -0.6000000000000388356, 2.500000000000000000, 3.983716857408420964 ) ) ;
#60538=CARTESIAN_POINT ( 'NONE',  ( 16.98713586915526008, -1.503435535905108811, -5.629434499184605478 ) ) ;
#60539=EDGE_CURVE ( 'NONE', #99244, #93665, #52638, .T. ) ;
#60540=CIRCLE ( 'NONE', #56297, 0.06509327318403745899 ) ;
#60541=VERTEX_POINT ( 'NONE', #32397 ) ;
#60542=AXIS2_PLACEMENT_3D ( 'NONE', #105191, #112456, #44335 ) ;
#60543=AXIS2_PLACEMENT_3D ( 'NONE', #55114, #95684, #5351 ) ;
#60544=ORIENTED_EDGE ( 'NONE', *, *, #11419, .F. ) ;
#60545=ORIENTED_EDGE ( 'NONE', *, *, #106009, .F. ) ;
#60546=DIRECTION ( 'NONE',  ( 0.000000000000000000, 0.000000000000000000, 1.000000000000000000 ) ) ;
#60547=PLANE ( 'NONE',  #104350 ) ;
#60548=DIRECTION ( 'NONE',  ( 0.000000000000000000, 0.000000000000000000, 1.000000000000000000 ) ) ;
#60549=FACE_BOUND ( 'NONE', #35515, .T. ) ;
#60550=ORIENTED_EDGE ( 'NONE', *, *, #28645, .T. ) ;
#60551=AXIS2_PLACEMENT_3D ( 'NONE', #102231, #14463, #125085 ) ;
#60552=DIRECTION ( 'NONE',  ( 0.000000000000000000, 1.000000000000000000, 0.000000000000000000 ) ) ;
#60553=DIRECTION ( 'NONE',  ( -4.274815082592931898E-19, -0.9999939076577903929, -0.003490651415223739937 ) ) ;
#60554=ORIENTED_EDGE ( 'NONE', *, *, #116220, .F. ) ;
#60555=CARTESIAN_POINT ( 'NONE',  ( -7.500000000000013323, 2.500000000000000000, 5.122947341949749323 ) ) ;
#60556=DIRECTION ( 'NONE',  ( 0.000000000000000000, 0.000000000000000000, -1.000000000000000000 ) ) ;
#60557=VECTOR ( 'NONE', #77411, 1000.000000000000000 ) ;
#60558=CARTESIAN_POINT ( 'NONE',  ( 6.249999999999930722, 2.500000000000000000, -1.472243186433550122 ) ) ;
#60559=DIRECTION ( 'NONE',  ( 0.000000000000000000, 1.000000000000000000, 0.000000000000000000 ) ) ;
#60560=DIRECTION ( 'NONE',  ( 0.000000000000000000, 1.000000000000000000, 0.000000000000000000 ) ) ;
#60561=DIRECTION ( 'NONE',  ( -0.000000000000000000, 1.000000000000000000, -0.000000000000000000 ) ) ;
#60562=DIRECTION ( 'NONE',  ( 0.000000000000000000, 0.000000000000000000, -1.000000000000000000 ) ) ;
#60563=EDGE_LOOP ( 'NONE', ( #81977, #36599 ) ) ;
#60564=ORIENTED_EDGE ( 'NONE', *, *, #43732, .F. ) ;
#60565=ORIENTED_EDGE ( 'NONE', *, *, #107661, .F. ) ;
#60566=ORIENTED_EDGE ( 'NONE', *, *, #41056, .F. ) ;
#60567=AXIS2_PLACEMENT_3D ( 'NONE', #51265, #29669, #851 ) ;
#60568=FACE_OUTER_BOUND ( 'NONE', #115950, .T. ) ;
#60569=DIRECTION ( 'NONE',  ( 0.000000000000000000, 1.000000000000000000, 0.000000000000000000 ) ) ;
#60570=ORIENTED_EDGE ( 'NONE', *, *, #41608, .T. ) ;
#60571=FACE_BOUND ( 'NONE', #88839, .T. ) ;
#60572=CARTESIAN_POINT ( 'NONE',  ( -4.600000000000024514, 2.500000000000000000, 5.022947341949748790 ) ) ;
#60573=EDGE_CURVE ( 'NONE', #39657, #46373, #1601, .T. ) ;
#60574=LINE ( 'NONE', #37842, #42925 ) ;
#60575=LINE ( 'NONE', #40940, #59610 ) ;
#60576=EDGE_CURVE ( 'NONE', #129477, #47052, #61841, .T. ) ;
#60577=DIRECTION ( 'NONE',  ( 0.000000000000000000, -0.9999939076577903929, 0.003490651415223739937 ) ) ;
#60578=DIRECTION ( 'NONE',  ( 0.000000000000000000, 1.000000000000000000, 0.000000000000000000 ) ) ;
#60579=DIRECTION ( 'NONE',  ( -4.274815082592931898E-19, -0.9999939076577903929, -0.003490651415223739937 ) ) ;
#60580=DIRECTION ( 'NONE',  ( 0.000000000000000000, 0.000000000000000000, 1.000000000000000000 ) ) ;
#60582=FACE_OUTER_BOUND ( 'NONE', #36620, .T. ) ;
#60583=VERTEX_POINT ( 'NONE', #112219 ) ;
#60584=EDGE_CURVE ( 'NONE', #7881, #125498, #13752, .T. ) ;
#60585=EDGE_LOOP ( 'NONE', ( #19352, #19022 ) ) ;
#60586=VERTEX_POINT ( 'NONE', #42861 ) ;
#60587=VERTEX_POINT ( 'NONE', #2912 ) ;
#60588=ORIENTED_EDGE ( 'NONE', *, *, #80197, .T. ) ;
#60589=ORIENTED_EDGE ( 'NONE', *, *, #51343, .F. ) ;
#60590=CARTESIAN_POINT ( 'NONE',  ( -4.350000000000027178, 12.50000000000000000, -6.148780366869526226 ) ) ;
#60591=AXIS2_PLACEMENT_3D ( 'NONE', #15646, #128876, #80401 ) ;
#60592=EDGE_LOOP ( 'NONE', ( #92899, #21920 ) ) ;
#60593=CIRCLE ( 'NONE', #6256, 0.1000000000000002554 ) ;
#60594=DIRECTION ( 'NONE',  ( 0.000000000000000000, 0.000000000000000000, -1.000000000000000000 ) ) ;
#60595=AXIS2_PLACEMENT_3D ( 'NONE', #36395, #57958, #117475 ) ;
#60597=CARTESIAN_POINT ( 'NONE',  ( -11.69999999999999929, 12.50000000000000000, 1.734723475976807094E-15 ) ) ;
#60598=CARTESIAN_POINT ( 'NONE',  ( -4.350000000000027178, 2.500000000000000000, -6.148780366869526226 ) ) ;
#60599=CIRCLE ( 'NONE', #114846, 0.1000000000000000056 ) ;
#60600=ORIENTED_EDGE ( 'NONE', *, *, #89790, .F. ) ;
#60601=FACE_OUTER_BOUND ( 'NONE', #78699, .T. ) ;
#60602=CONICAL_SURFACE ( 'NONE', #119073, 0.09999999999999982514, 0.003490658503988666988 ) ;
#60603=CIRCLE ( 'NONE', #81429, 0.1000000000000000056 ) ;
#60604=ORIENTED_EDGE ( 'NONE', *, *, #93804, .T. ) ;
#60605=ORIENTED_EDGE ( 'NONE', *, *, #126097, .T. ) ;
#60606=CARTESIAN_POINT ( 'NONE',  ( 14.54999999999989235, 12.50000000000000000, -2.165063509461101710 ) ) ;
#60607=CARTESIAN_POINT ( 'NONE',  ( 3.349999999999945466, 2.500000000000000000, -7.088010851410853519 ) ) ;
#60608=DIRECTION ( 'NONE',  ( 0.000000000000000000, 1.000000000000000000, 0.000000000000000000 ) ) ;
#60609=EDGE_LOOP ( 'NONE', ( #30948, #26890, #122163, #114453 ) ) ;
#60610=EDGE_LOOP ( 'NONE', ( #59012, #80153, #13024, #126310 ) ) ;
#60611=ADVANCED_FACE ( 'NONE', ( #101754 ), #62486, .T. ) ;
#60612=CARTESIAN_POINT ( 'NONE',  ( 1.249999999999988454, 2.500000000000000000, 2.165063509461097713 ) ) ;
#60613=DIRECTION ( 'NONE',  ( 0.000000000000000000, 0.000000000000000000, 1.000000000000000000 ) ) ;
#60614=CARTESIAN_POINT ( 'NONE',  ( -3.750000000000027534, 12.50000000000000000, 2.857883832488649301 ) ) ;
#60615=DIRECTION ( 'NONE',  ( 0.000000000000000000, -0.9999939076577903929, 0.003490651415223739937 ) ) ;
#60616=ORIENTED_EDGE ( 'NONE', *, *, #121482, .F. ) ;
#60617=DIRECTION ( 'NONE',  ( -4.274815082592931898E-19, -0.9999939076577903929, -0.003490651415223739937 ) ) ;
#60618=ORIENTED_EDGE ( 'NONE', *, *, #117330, .T. ) ;
#60619=CARTESIAN_POINT ( 'NONE',  ( 1.899999999999951283, 2.500000000000000000, 0.3464101615137736845 ) ) ;
#60620=CIRCLE ( 'NONE', #91903, 0.1000000000000000056 ) ;
#60621=CIRCLE ( 'NONE', #39784, 0.1000000000000000056 ) ;
#60622=ORIENTED_EDGE ( 'NONE', *, *, #16024, .T. ) ;
#60623=FACE_OUTER_BOUND ( 'NONE', #686, .T. ) ;
#60624=CARTESIAN_POINT ( 'NONE',  ( 48.81613170260295220, -3.619496531216669588, 4.312669415525522965 ) ) ;
#60625=DIRECTION ( 'NONE',  ( -0.000000000000000000, 1.000000000000000000, -0.000000000000000000 ) ) ;
#60626=EDGE_CURVE ( 'NONE', #65247, #123233, #53306, .T. ) ;
#60627=EDGE_CURVE ( 'NONE', #18103, #3294, #105718, .T. ) ;
#60628=CARTESIAN_POINT ( 'NONE',  ( 12.04999999999990834, 2.500000000000000000, -2.165063509461101710 ) ) ;
#60629=EDGE_LOOP ( 'NONE', ( #121931, #84454 ) ) ;
#60630=AXIS2_PLACEMENT_3D ( 'NONE', #57702, #97612, #7933 ) ;
#60631=CARTESIAN_POINT ( 'NONE',  ( -11.89999999999999503, 2.500000000000000000, 3.983716857408420076 ) ) ;
#60632=CARTESIAN_POINT ( 'NONE',  ( 0.6499999999999561684, 12.50000000000000000, -2.446380397790840266 ) ) ;
#60633=EDGE_LOOP ( 'NONE', ( #127318, #94706, #72592, #116714 ) ) ;
#60634=VERTEX_POINT ( 'NONE', #122674 ) ;
#60635=ADVANCED_FACE ( 'NONE', ( #20619 ), #65994, .T. ) ;
#60636=VERTEX_POINT ( 'NONE', #72933 ) ;
#60637=LINE ( 'NONE', #42276, #1868 ) ;
#60638=DIRECTION ( 'NONE',  ( 0.000000000000000000, 0.000000000000000000, 1.000000000000000000 ) ) ;
#60639=DIRECTION ( 'NONE',  ( -0.000000000000000000, -1.000000000000000000, -0.000000000000000000 ) ) ;
#60640=AXIS2_PLACEMENT_3D ( 'NONE', #55694, #50245, #28670 ) ;
#60641=DIRECTION ( 'NONE',  ( 0.000000000000000000, 0.000000000000000000, 1.000000000000000000 ) ) ;
#60642=FACE_OUTER_BOUND ( 'NONE', #85993, .T. ) ;
#60643=AXIS2_PLACEMENT_3D ( 'NONE', #127144, #38113, #85269 ) ;
#60644=CARTESIAN_POINT ( 'NONE',  ( -1.250000000000001554, 2.500000000000000000, 6.495190528383297135 ) ) ;
#60645=DIRECTION ( 'NONE',  ( -4.274815082592931898E-19, -0.9999939076577903929, -0.003490651415223739937 ) ) ;
#60646=DIRECTION ( 'NONE',  ( -4.274815082592931898E-19, -0.9999939076577903929, -0.003490651415223739937 ) ) ;
#60647=VECTOR ( 'NONE', #36759, 1000.000000000000000 ) ;
#60648=CONICAL_SURFACE ( 'NONE', #35511, 0.09999999999999982514, 0.003490658503988666988 ) ;
#60649=VERTEX_POINT ( 'NONE', #10755 ) ;
#60650=CONICAL_SURFACE ( 'NONE', #16784, 0.1000000000000002554, 0.003490658503988666988 ) ;
#60651=DIRECTION ( 'NONE',  ( -0.000000000000000000, 1.000000000000000000, -0.000000000000000000 ) ) ;
#60652=CARTESIAN_POINT ( 'NONE',  ( 12.09999999999990550, 2.500000000000000000, 5.022947341949748790 ) ) ;
#60653=LINE ( 'NONE', #88805, #61055 ) ;
#60654=PLANE ( 'NONE',  #73001 ) ;
#60655=EDGE_LOOP ( 'NONE', ( #69774, #125883, #6004, #122950 ) ) ;
#60656=DIRECTION ( 'NONE',  ( -0.000000000000000000, 1.000000000000000000, -0.000000000000000000 ) ) ;
#60657=EDGE_CURVE ( 'NONE', #60435, #53973, #99466, .T. ) ;
#60658=DIRECTION ( 'NONE',  ( 0.000000000000000000, 1.000000000000000000, 0.000000000000000000 ) ) ;
#60659=DIRECTION ( 'NONE',  ( 0.000000000000000000, 0.000000000000000000, 1.000000000000000000 ) ) ;
#60661=ADVANCED_FACE ( 'NONE', ( #63106 ), #57696, .T. ) ;
#60662=EDGE_CURVE ( 'NONE', #121281, #25124, #55628, .T. ) ;
#60663=EDGE_LOOP ( 'NONE', ( #99352, #109817 ) ) ;
#60664=DIRECTION ( 'NONE',  ( 0.000000000000000000, 0.000000000000000000, -1.000000000000000000 ) ) ;
#60665=EDGE_LOOP ( 'NONE', ( #90424, #121582 ) ) ;
#60666=ORIENTED_EDGE ( 'NONE', *, *, #95915, .F. ) ;
#60667=CARTESIAN_POINT ( 'NONE',  ( -11.64999999999999680, 12.50000000000000000, -2.857883832488649745 ) ) ;
#60668=EDGE_CURVE ( 'NONE', #111704, #90001, #70206, .T. ) ;
#60669=CIRCLE ( 'NONE', #35626, 0.1000000000000000472 ) ;
#60670=EDGE_CURVE ( 'NONE', #82618, #90496, #74223, .T. ) ;
#60671=ADVANCED_FACE ( 'NONE', ( #124614 ), #72277, .T. ) ;
#60672=CARTESIAN_POINT ( 'NONE',  ( 20.25366426269120268, 2.573118374676206521, -4.179292740213720769 ) ) ;
#60673=CARTESIAN_POINT ( 'NONE',  ( 1.449999999999949551, 12.50000000000000000, 6.776507416713035248 ) ) ;
#60674=CARTESIAN_POINT ( 'NONE',  ( -10.40000000000000213, 2.500000000000000000, -5.022947341949749678 ) ) ;
#60675=ORIENTED_EDGE ( 'NONE', *, *, #67722, .T. ) ;
#60676=AXIS2_PLACEMENT_3D ( 'NONE', #55179, #63063, #102980 ) ;
#60677=AXIS2_PLACEMENT_3D ( 'NONE', #24468, #31715, #13344 ) ;
#60678=ADVANCED_FACE ( 'NONE', ( #26419 ), #84680, .T. ) ;
#60680=ORIENTED_EDGE ( 'NONE', *, *, #97497, .T. ) ;
#60681=DIRECTION ( 'NONE',  ( 0.000000000000000000, 1.000000000000000000, 0.000000000000000000 ) ) ;
#60683=EDGE_CURVE ( 'NONE', #9406, #46747, #104945, .T. ) ;
#60684=CARTESIAN_POINT ( 'NONE',  ( 16.68631762705459565, -1.607367762587846860, 5.954228785335645924 ) ) ;
#60685=EDGE_CURVE ( 'NONE', #109850, #61759, #34961, .T. ) ;
#60686=VERTEX_POINT ( 'NONE', #44773 ) ;
#60687=VECTOR ( 'NONE', #16500, 1000.000000000000000 ) ;
#60688=EDGE_LOOP ( 'NONE', ( #75859, #34303, #6087, #118816 ) ) ;
#60689=ORIENTED_EDGE ( 'NONE', *, *, #123662, .T. ) ;
#60690=ORIENTED_EDGE ( 'NONE', *, *, #118861, .F. ) ;
#60691=CARTESIAN_POINT ( 'NONE',  ( 12.09999999999990195, 12.50000000000000000, 0.6928203230275494784 ) ) ;
#60692=CARTESIAN_POINT ( 'NONE',  ( 15.22989033483572996, 1.499999999999839462, 7.180069493258938174 ) ) ;
#60693=FACE_OUTER_BOUND ( 'NONE', #73016, .T. ) ;
#60694=FACE_BOUND ( 'NONE', #113638, .T. ) ;
#60695=CARTESIAN_POINT ( 'NONE',  ( 6.449999999999931788, 2.500000000000000000, 6.248780366869520542 ) ) ;
#60697=FACE_OUTER_BOUND ( 'NONE', #119443, .T. ) ;
#60698=CARTESIAN_POINT ( 'NONE',  ( -2.950000000000029932, 2.500000000000000000, -2.165063509461101710 ) ) ;
#60699=CARTESIAN_POINT ( 'NONE',  ( 8.349999999999919709, 2.500000000000000000, -2.757883832488654097 ) ) ;
#60700=CARTESIAN_POINT ( 'NONE',  ( -10.65000000000000391, 2.500000000000000000, -2.611473670974873595 ) ) ;
#60701=CARTESIAN_POINT ( 'NONE',  ( 9.999999999999916511, 12.50000000000000000, -0.6928203230275541413 ) ) ;
#60702=CARTESIAN_POINT ( 'NONE',  ( -1.650000000000034772, 12.50000000000000000, 2.230156782645134950 ) ) ;
#60703=ORIENTED_EDGE ( 'NONE', *, *, #33682, .T. ) ;
#60704=ORIENTED_EDGE ( 'NONE', *, *, #51468, .F. ) ;
#60705=ORIENTED_EDGE ( 'NONE', *, *, #30718, .F. ) ;
#60706=EDGE_LOOP ( 'NONE', ( #18864, #10002, #119136, #26820 ) ) ;
#60707=CARTESIAN_POINT ( 'NONE',  ( 2.899999999999944844, 12.50000000000000000, 3.637306695894644726 ) ) ;
#60708=PLANE ( 'NONE',  #19499 ) ;
#60709=ORIENTED_EDGE ( 'NONE', *, *, #98487, .F. ) ;
#60710=FACE_BOUND ( 'NONE', #29005, .T. ) ;
#60711=CIRCLE ( 'NONE', #94148, 0.1000000000000002554 ) ;
#60712=CARTESIAN_POINT ( 'NONE',  ( 8.149999999999920419, 12.50000000000000000, -1.883746621131363375 ) ) ;
#60713=EDGE_CURVE ( 'NONE', #10391, #60441, #109926, .T. ) ;
#60714=ORIENTED_EDGE ( 'NONE', *, *, #64480, .T. ) ;
#60715=LINE ( 'NONE', #109143, #11205 ) ;
#60716=CARTESIAN_POINT ( 'NONE',  ( 8.099999999999921485, 2.500000000000000000, 0.2464101615137735679 ) ) ;
#60717=DIRECTION ( 'NONE',  ( 0.000000000000000000, -0.9999939076577903929, 0.003490651415223739937 ) ) ;
#60718=DIRECTION ( 'NONE',  ( -0.000000000000000000, -1.000000000000000000, -0.000000000000000000 ) ) ;
#60719=ORIENTED_EDGE ( 'NONE', *, *, #73193, .F. ) ;
#60720=CARTESIAN_POINT ( 'NONE',  ( -11.44999999999999751, 2.500000000000000000, 6.048780366869521252 ) ) ;
#60721=EDGE_CURVE ( 'NONE', #56093, #27833, #74870, .T. ) ;
#60722=AXIS2_PLACEMENT_3D ( 'NONE', #55654, #26201, #36680 ) ;
#60723=ORIENTED_EDGE ( 'NONE', *, *, #109906, .F. ) ;
#60724=ORIENTED_EDGE ( 'NONE', *, *, #96682, .T. ) ;
#60725=DIRECTION ( 'NONE',  ( -0.000000000000000000, 1.000000000000000000, -0.000000000000000000 ) ) ;
#60726=DIRECTION ( 'NONE',  ( 0.000000000000000000, 0.000000000000000000, -1.000000000000000000 ) ) ;
#60727=VERTEX_POINT ( 'NONE', #116071 ) ;
#60728=LINE ( 'NONE', #117185, #114313 ) ;
#60729=CONICAL_SURFACE ( 'NONE', #66956, 0.1000000000000000472, 0.003490658503988666988 ) ;
#60730=DIRECTION ( 'NONE',  ( 0.000000000000000000, 0.000000000000000000, 1.000000000000000000 ) ) ;
#60731=CARTESIAN_POINT ( 'NONE',  ( -0.6000000000000383915, 12.50000000000000000, -4.611443907251939756 ) ) ;
#60732=DIRECTION ( 'NONE',  ( 0.000000000000000000, 1.000000000000000000, 0.000000000000000000 ) ) ;
#60733=VECTOR ( 'NONE', #30124, 1000.000000000000000 ) ;
#60734=VERTEX_POINT ( 'NONE', #65680 ) ;
#60735=FACE_OUTER_BOUND ( 'NONE', #35721, .T. ) ;
#60736=VERTEX_POINT ( 'NONE', #44113 ) ;
#60737=DIRECTION ( 'NONE',  ( -0.000000000000000000, -1.000000000000000000, -0.000000000000000000 ) ) ;
#60738=ORIENTED_EDGE ( 'NONE', *, *, #60364, .T. ) ;
#60739=DIRECTION ( 'NONE',  ( 0.000000000000000000, 0.000000000000000000, -1.000000000000000000 ) ) ;
#60740=ORIENTED_EDGE ( 'NONE', *, *, #86057, .T. ) ;
#60741=DIRECTION ( 'NONE',  ( -0.000000000000000000, -1.000000000000000000, -0.000000000000000000 ) ) ;
#60742=CARTESIAN_POINT ( 'NONE',  ( -0.2000000000000404232, 2.500000000000000000, 3.883716857408421319 ) ) ;
#60743=CARTESIAN_POINT ( 'NONE',  ( 8.949999999999917577, 2.500000000000000000, 6.248780366869520542 ) ) ;
#60744=FACE_OUTER_BOUND ( 'NONE', #36915, .T. ) ;
#60745=CARTESIAN_POINT ( 'NONE',  ( -10.60000000000000142, 2.500000000000000000, -0.3464101615137782364 ) ) ;
#60746=EDGE_LOOP ( 'NONE', ( #6921, #32079, #19496, #11388 ) ) ;
#60747=ORIENTED_EDGE ( 'NONE', *, *, #74092, .T. ) ;
#60748=EDGE_CURVE ( 'NONE', #52226, #60021, #7498, .T. ) ;
#60749=ORIENTED_EDGE ( 'NONE', *, *, #111327, .F. ) ;
#60751=CARTESIAN_POINT ( 'NONE',  ( 1.449999999999951328, 12.50000000000000000, 2.511473670974873507 ) ) ;
#60752=DIRECTION ( 'NONE',  ( -0.000000000000000000, 1.000000000000000000, -0.000000000000000000 ) ) ;
#60753=VERTEX_POINT ( 'NONE', #14630 ) ;
#60754=ORIENTED_EDGE ( 'NONE', *, *, #108778, .T. ) ;
#60755=VERTEX_POINT ( 'NONE', #73558 ) ;
#60756=AXIS2_PLACEMENT_3D ( 'NONE', #18732, #68471, #78964 ) ;
#60757=DIRECTION ( 'NONE',  ( 0.000000000000000000, 1.000000000000000000, 0.000000000000000000 ) ) ;
#60758=EDGE_LOOP ( 'NONE', ( #93942, #30521, #100971, #6871 ) ) ;
#60759=DIRECTION ( 'NONE',  ( 0.000000000000000000, 0.000000000000000000, -1.000000000000000000 ) ) ;
#60760=EDGE_CURVE ( 'NONE', #15697, #119380, #126647, .T. ) ;
#60762=FACE_OUTER_BOUND ( 'NONE', #83837, .T. ) ;
#60763=DIRECTION ( 'NONE',  ( 0.000000000000000000, 0.000000000000000000, -1.000000000000000000 ) ) ;
#60764=DIRECTION ( 'NONE',  ( 0.000000000000000000, 0.000000000000000000, 1.000000000000000000 ) ) ;
#60766=FACE_OUTER_BOUND ( 'NONE', #121659, .T. ) ;
#60767=EDGE_CURVE ( 'NONE', #12520, #77015, #30523, .T. ) ;
#60768=ADVANCED_FACE ( 'NONE', ( #85951 ), #34317, .T. ) ;
#60769=LINE ( 'NONE', #39861, #49989 ) ;
#60770=EDGE_LOOP ( 'NONE', ( #92416, #37513, #16951, #96375 ) ) ;
#60771=EDGE_LOOP ( 'NONE', ( #116409, #108219, #39749, #3474 ) ) ;
#60772=DIRECTION ( 'NONE',  ( 0.000000000000000000, 1.000000000000000000, 0.000000000000000000 ) ) ;
#60773=EDGE_CURVE ( 'NONE', #125197, #109336, #107855, .T. ) ;
#60775=ORIENTED_EDGE ( 'NONE', *, *, #31810, .T. ) ;
#60776=ORIENTED_EDGE ( 'NONE', *, *, #108373, .T. ) ;
#60777=ADVANCED_FACE ( 'NONE', ( #65017 ), #4170, .T. ) ;
#60779=DIRECTION ( 'NONE',  ( 0.000000000000000000, 1.000000000000000000, 0.000000000000000000 ) ) ;
#60780=DIRECTION ( 'NONE',  ( 0.000000000000000000, 0.000000000000000000, -1.000000000000000000 ) ) ;
#60781=CARTESIAN_POINT ( 'NONE',  ( 10.64999999999990976, 2.500000000000000000, 2.611473670974873151 ) ) ;
#60782=DIRECTION ( 'NONE',  ( 0.000000000000000000, 0.000000000000000000, -1.000000000000000000 ) ) ;
#60783=CARTESIAN_POINT ( 'NONE',  ( 5.199999999999933564, 12.50000000000000000, 3.918623584224382839 ) ) ;
#60784=LINE ( 'NONE', #1211, #42752 ) ;
#60785=CARTESIAN_POINT ( 'NONE',  ( -9.350000000000006750, 2.500000000000000000, -1.718653347947325827 ) ) ;
#60787=CIRCLE ( 'NONE', #69170, 0.06509327318403745899 ) ;
#60788=ORIENTED_EDGE ( 'NONE', *, *, #36635, .T. ) ;
#60790=ORIENTED_EDGE ( 'NONE', *, *, #76784, .F. ) ;
#60791=EDGE_CURVE ( 'NONE', #19759, #21177, #114148, .T. ) ;
#60792=ORIENTED_EDGE ( 'NONE', *, *, #119046, .F. ) ;
#60793=VERTEX_POINT ( 'NONE', #13993 ) ;
#60794=EDGE_LOOP ( 'NONE', ( #15929, #103235 ) ) ;
#60795=CARTESIAN_POINT ( 'NONE',  ( 2.699999999999945555, 2.500000000000000000, 3.983716857408420076 ) ) ;
#60796=CARTESIAN_POINT ( 'NONE',  ( -2.300000000000033573, 12.50000000000000000, 4.676537180435972552 ) ) ;
#60797=AXIS2_PLACEMENT_3D ( 'NONE', #58734, #97362, #58094 ) ;
#60798=VERTEX_POINT ( 'NONE', #86607 ) ;
#60799=CARTESIAN_POINT ( 'NONE',  ( -10.40000000000000213, 12.50000000000000000, -5.022947341949749678 ) ) ;
#60800=EDGE_CURVE ( 'NONE', #39517, #34970, #68137, .T. ) ;
#60801=FACE_OUTER_BOUND ( 'NONE', #74611, .T. ) ;
#60802=CARTESIAN_POINT ( 'NONE',  ( 0.6499999999999561684, 12.50000000000000000, -2.511473670974877948 ) ) ;
#60803=ORIENTED_EDGE ( 'NONE', *, *, #85329, .T. ) ;
#60804=EDGE_CURVE ( 'NONE', #31864, #97088, #28449, .T. ) ;
#60805=DIRECTION ( 'NONE',  ( 0.000000000000000000, 1.000000000000000000, 0.000000000000000000 ) ) ;
#60806=ADVANCED_FACE ( 'NONE', ( #4815 ), #38937, .T. ) ;
#60807=CARTESIAN_POINT ( 'NONE',  ( -1.250000000000037970, 12.50000000000000000, 7.188010851410848723 ) ) ;
#60808=VECTOR ( 'NONE', #62116, 1000.000000000000000 ) ;
#60809=ORIENTED_EDGE ( 'NONE', *, *, #125520, .T. ) ;
#60810=VECTOR ( 'NONE', #105758, 1000.000000000000000 ) ;
#60811=ORIENTED_EDGE ( 'NONE', *, *, #69034, .T. ) ;
#60812=ORIENTED_EDGE ( 'NONE', *, *, #74092, .F. ) ;
#60813=EDGE_LOOP ( 'NONE', ( #3502, #74401, #28300, #83624 ) ) ;
#60814=CARTESIAN_POINT ( 'NONE',  ( 10.79999999999991367, 2.500000000000000000, 0.09999999999999761857 ) ) ;
#60815=EDGE_CURVE ( 'NONE', #19198, #50142, #69543, .T. ) ;
#60817=VECTOR ( 'NONE', #10291, 1000.000000000000000 ) ;
#60818=ADVANCED_FACE ( 'NONE', ( #59761 ), #80778, .T. ) ;
#60819=DIRECTION ( 'NONE',  ( 0.000000000000000000, 0.000000000000000000, 1.000000000000000000 ) ) ;
#60820=DIRECTION ( 'NONE',  ( 0.000000000000000000, 1.000000000000000000, 0.000000000000000000 ) ) ;
#60821=EDGE_CURVE ( 'NONE', #100917, #47413, #20124, .T. ) ;
#60822=AXIS2_PLACEMENT_3D ( 'NONE', #71008, #113496, #21915 ) ;
#60823=CARTESIAN_POINT ( 'NONE',  ( -8.550000000000007816, 2.500000000000000000, 6.148780366869520009 ) ) ;
#60824=ORIENTED_EDGE ( 'NONE', *, *, #116079, .T. ) ;
#60825=DIRECTION ( 'NONE',  ( 0.000000000000000000, 0.000000000000000000, 1.000000000000000000 ) ) ;
#60826=DIRECTION ( 'NONE',  ( -0.000000000000000000, -1.000000000000000000, -0.000000000000000000 ) ) ;
#60827=DIRECTION ( 'NONE',  ( 0.000000000000000000, 0.000000000000000000, -1.000000000000000000 ) ) ;
#60828=FACE_OUTER_BOUND ( 'NONE', #120467, .T. ) ;
#60829=EDGE_CURVE ( 'NONE', #62165, #31928, #87016, .T. ) ;
#60830=ORIENTED_EDGE ( 'NONE', *, *, #88120, .F. ) ;
#60831=EDGE_CURVE ( 'NONE', #90527, #113115, #78754, .T. ) ;
#60832=VERTEX_POINT ( 'NONE', #99670 ) ;
#60834=CARTESIAN_POINT ( 'NONE',  ( -0.8000000000000381251, 12.50000000000000000, 4.330127018922196314 ) ) ;
#60835=DIRECTION ( 'NONE',  ( -0.000000000000000000, -1.000000000000000000, -0.000000000000000000 ) ) ;
#60836=FACE_BOUND ( 'NONE', #103328, .T. ) ;
#60837=PLANE ( 'NONE',  #105725 ) ;
#60838=CARTESIAN_POINT ( 'NONE',  ( 13.14999999999989733, 2.500000000000000000, -1.918653347947325782 ) ) ;
#60839=CARTESIAN_POINT ( 'NONE',  ( -5.850000000000021849, 2.500000000000000000, -1.372243186433550033 ) ) ;
#60840=CIRCLE ( 'NONE', #54481, 0.06509327318403745899 ) ;
#60841=CIRCLE ( 'NONE', #4375, 0.06509327318403743123 ) ;
#60842=DIRECTION ( 'NONE',  ( 0.000000000000000000, 0.000000000000000000, 1.000000000000000000 ) ) ;
#60843=VECTOR ( 'NONE', #42919, 1000.000000000000000 ) ;
#60844=DIRECTION ( 'NONE',  ( 0.000000000000000000, 1.000000000000000000, 0.000000000000000000 ) ) ;
#60845=DIRECTION ( 'NONE',  ( -0.000000000000000000, -1.000000000000000000, -0.000000000000000000 ) ) ;
#60846=ORIENTED_EDGE ( 'NONE', *, *, #10373, .T. ) ;
#60847=DIRECTION ( 'NONE',  ( -0.000000000000000000, 1.000000000000000000, -0.000000000000000000 ) ) ;
#60848=AXIS2_PLACEMENT_3D ( 'NONE', #125674, #75937, #28144 ) ;
#60849=CARTESIAN_POINT ( 'NONE',  ( 3.299999999999944755, 12.50000000000000000, -0.06509327318403980434 ) ) ;
#60850=VERTEX_POINT ( 'NONE', #28998 ) ;
#60851=ORIENTED_EDGE ( 'NONE', *, *, #8362, .F. ) ;
#60852=VECTOR ( 'NONE', #2291, 1000.000000000000000 ) ;
#60853=DIRECTION ( 'NONE',  ( -0.000000000000000000, 1.000000000000000000, -0.000000000000000000 ) ) ;
#60854=DIRECTION ( 'NONE',  ( 0.000000000000000000, 0.000000000000000000, -1.000000000000000000 ) ) ;
#60855=FACE_BOUND ( 'NONE', #82065, .T. ) ;
#60856=CARTESIAN_POINT ( 'NONE',  ( -9.600000000000006750, 12.50000000000000000, 0.6928203230275494784 ) ) ;
#60857=DIRECTION ( 'NONE',  ( 0.000000000000000000, 0.000000000000000000, -1.000000000000000000 ) ) ;
#60858=EDGE_CURVE ( 'NONE', #12489, #90022, #66083, .T. ) ;
#60859=EDGE_LOOP ( 'NONE', ( #86665, #123827 ) ) ;
#60860=CARTESIAN_POINT ( 'NONE',  ( -11.25000000000000178, 2.500000000000000000, -1.472243186433546125 ) ) ;
#60862=ORIENTED_EDGE ( 'NONE', *, *, #46249, .T. ) ;
#60863=LINE ( 'NONE', #61528, #51137 ) ;
#60864=CARTESIAN_POINT ( 'NONE',  ( -8.100000000000013856, 12.50000000000000000, -4.611443907251939756 ) ) ;
#60865=EDGE_CURVE ( 'NONE', #103728, #64891, #99557, .T. ) ;
#60866=CONICAL_SURFACE ( 'NONE', #118167, 0.1000000000000002554, 0.003490658503988666988 ) ;
#60867=PLANE ( 'NONE',  #107140 ) ;
#60868=DIRECTION ( 'NONE',  ( 0.000000000000000000, 0.000000000000000000, -1.000000000000000000 ) ) ;
#60869=AXIS2_PLACEMENT_3D ( 'NONE', #47759, #118416, #87659 ) ;
#60870=AXIS2_PLACEMENT_3D ( 'NONE', #95377, #126119, #25328 ) ;
#60872=LINE ( 'NONE', #100778, #88468 ) ;
#60873=DIRECTION ( 'NONE',  ( 0.000000000000000000, 0.000000000000000000, 1.000000000000000000 ) ) ;
#60874=CARTESIAN_POINT ( 'NONE',  ( 10.84999999999991260, 2.500000000000000000, -2.065063509461102065 ) ) ;
#60875=EDGE_LOOP ( 'NONE', ( #22967, #83257, #67885, #10434 ) ) ;
#60876=ORIENTED_EDGE ( 'NONE', *, *, #60670, .F. ) ;
#60877=FACE_OUTER_BOUND ( 'NONE', #86847, .T. ) ;
#60878=CIRCLE ( 'NONE', #108894, 0.06509327318403745899 ) ;
#60879=ORIENTED_EDGE ( 'NONE', *, *, #105898, .F. ) ;
#60880=DIRECTION ( 'NONE',  ( 0.000000000000000000, -0.000000000000000000, 1.000000000000000000 ) ) ;
#60881=VECTOR ( 'NONE', #49202, 1000.000000000000000 ) ;
#60882=FACE_OUTER_BOUND ( 'NONE', #81217, .T. ) ;
#60883=CARTESIAN_POINT ( 'NONE',  ( -13.94999999999998685, 2.500000000000000000, 1.818653347947325472 ) ) ;
#60884=ORIENTED_EDGE ( 'NONE', *, *, #69631, .F. ) ;
#60886=FACE_OUTER_BOUND ( 'NONE', #26311, .T. ) ;
#60887=DIRECTION ( 'NONE',  ( -0.000000000000000000, -1.000000000000000000, -0.000000000000000000 ) ) ;
#60888=CARTESIAN_POINT ( 'NONE',  ( 12.09999999999990550, 12.50000000000000000, 4.330127018922196314 ) ) ;
#60889=DIRECTION ( 'NONE',  ( -0.000000000000000000, 1.000000000000000000, -0.000000000000000000 ) ) ;
#60890=LINE ( 'NONE', #83756, #36902 ) ;
#60891=AXIS2_PLACEMENT_3D ( 'NONE', #78382, #79026, #89474 ) ;
#60892=ORIENTED_EDGE ( 'NONE', *, *, #46707, .T. ) ;
#60893=ORIENTED_EDGE ( 'NONE', *, *, #32174, .T. ) ;
#60894=LINE ( 'NONE', #2602, #64132 ) ;
#60895=ORIENTED_EDGE ( 'NONE', *, *, #99780, .F. ) ;
#60896=DIRECTION ( 'NONE',  ( -4.274815082592931898E-19, -0.9999939076577903929, -0.003490651415223739937 ) ) ;
#60897=ORIENTED_EDGE ( 'NONE', *, *, #63455, .T. ) ;
#60898=EDGE_LOOP ( 'NONE', ( #118257, #48481 ) ) ;
#60899=ORIENTED_EDGE ( 'NONE', *, *, #104987, .T. ) ;
#60900=CARTESIAN_POINT ( 'NONE',  ( 3.149999999999946176, 12.50000000000000000, -2.576566944158915184 ) ) ;
#60901=AXIS2_PLACEMENT_3D ( 'NONE', #50229, #99322, #9643 ) ;
#60902=DIRECTION ( 'NONE',  ( 0.000000000000000000, 1.000000000000000000, 0.000000000000000000 ) ) ;
#60903=EDGE_CURVE ( 'NONE', #18843, #72282, #36858, .T. ) ;
#60904=DIRECTION ( 'NONE',  ( -0.000000000000000000, 1.000000000000000000, -0.000000000000000000 ) ) ;
#60905=LINE ( 'NONE', #121118, #89049 ) ;
#60906=AXIS2_PLACEMENT_3D ( 'NONE', #116073, #123956, #95794 ) ;
#60907=CONICAL_SURFACE ( 'NONE', #33721, 0.09999999999999982514, 0.003490658503988666988 ) ;
#60908=DIRECTION ( 'NONE',  ( 0.000000000000000000, -0.9999939076577903929, 0.003490651415223739937 ) ) ;
#60909=CARTESIAN_POINT ( 'NONE',  ( -9.600000000000006750, 2.500000000000000000, 5.022947341949748790 ) ) ;
#60910=CARTESIAN_POINT ( 'NONE',  ( -13.94999999999998863, 2.500000000000000000, 2.511473670974877503 ) ) ;
#60911=DIRECTION ( 'NONE',  ( 0.000000000000000000, -0.000000000000000000, 1.000000000000000000 ) ) ;
#60912=EDGE_CURVE ( 'NONE', #25279, #52919, #19139, .T. ) ;
#60913=ADVANCED_FACE ( 'NONE', ( #76803 ), #107952, .T. ) ;
#60914=CARTESIAN_POINT ( 'NONE',  ( -11.89999999999999503, 2.500000000000000000, 4.776537180435972196 ) ) ;
#60915=VERTEX_POINT ( 'NONE', #49293 ) ;
#60916=EDGE_CURVE ( 'NONE', #10113, #12902, #70304, .T. ) ;
#60917=FACE_OUTER_BOUND ( 'NONE', #43708, .T. ) ;
#60918=EDGE_CURVE ( 'NONE', #54077, #30501, #55709, .T. ) ;
#60919=ORIENTED_EDGE ( 'NONE', *, *, #73660, .F. ) ;
#60920=ORIENTED_EDGE ( 'NONE', *, *, #106727, .T. ) ;
#60921=EDGE_CURVE ( 'NONE', #127834, #100677, #66954, .T. ) ;
#60922=CARTESIAN_POINT ( 'NONE',  ( -9.800000000000004263, 2.500000000000000000, -0.3464101615137783474 ) ) ;
#60923=LINE ( 'NONE', #30843, #61217 ) ;
#60924=LINE ( 'NONE', #128409, #83858 ) ;
#60925=CARTESIAN_POINT ( 'NONE',  ( 10.84999999999991260, 2.500000000000000000, -2.957883832488653830 ) ) ;
#60926=LINE ( 'NONE', #79925, #84549 ) ;
#60927=AXIS2_PLACEMENT_3D ( 'NONE', #45164, #106010, #107288 ) ;
#60928=DIRECTION ( 'NONE',  ( 0.000000000000000000, -0.000000000000000000, 1.000000000000000000 ) ) ;
#60929=ORIENTED_EDGE ( 'NONE', *, *, #71233, .T. ) ;
#60930=AXIS2_PLACEMENT_3D ( 'NONE', #51139, #723, #40685 ) ;
#60932=DIRECTION ( 'NONE',  ( 0.000000000000000000, -1.000000000000000000, 0.000000000000000000 ) ) ;
#60933=AXIS2_PLACEMENT_3D ( 'NONE', #92874, #34611, #81739 ) ;
#60934=ORIENTED_EDGE ( 'NONE', *, *, #91534, .F. ) ;
#60935=AXIS2_PLACEMENT_3D ( 'NONE', #31288, #100639, #10953 ) ;
#60936=CARTESIAN_POINT ( 'NONE',  ( 5.599999999999933031, 12.50000000000000000, -0.3464101615137783474 ) ) ;
#60937=ORIENTED_EDGE ( 'NONE', *, *, #48525, .F. ) ;
#60938=AXIS2_PLACEMENT_3D ( 'NONE', #58521, #7452, #8731 ) ;
#60939=EDGE_LOOP ( 'NONE', ( #82815, #7025 ) ) ;
#60940=DIRECTION ( 'NONE',  ( 0.000000000000000000, -0.9999939076577903929, 0.003490651415223739937 ) ) ;
#60941=DIRECTION ( 'NONE',  ( 0.000000000000000000, 0.000000000000000000, 1.000000000000000000 ) ) ;
#60942=DIRECTION ( 'NONE',  ( -0.000000000000000000, 1.000000000000000000, -0.000000000000000000 ) ) ;
#60943=DIRECTION ( 'NONE',  ( 0.000000000000000000, 0.000000000000000000, 1.000000000000000000 ) ) ;
#60944=FACE_OUTER_BOUND ( 'NONE', #51435, .T. ) ;
#60945=EDGE_LOOP ( 'NONE', ( #102343, #115092 ) ) ;
#60946=CARTESIAN_POINT ( 'NONE',  ( 2.699999999999947331, 12.50000000000000000, -4.611443907251940644 ) ) ;
#60947=CARTESIAN_POINT ( 'NONE',  ( 1.449999999999951772, 12.50000000000000000, -6.083687093685488989 ) ) ;
#60948=DIRECTION ( 'NONE',  ( 0.000000000000000000, 0.000000000000000000, 1.000000000000000000 ) ) ;
#60949=FACE_OUTER_BOUND ( 'NONE', #123446, .T. ) ;
#60950=CARTESIAN_POINT ( 'NONE',  ( -5.850000000000021849, 12.50000000000000000, -5.802370205355749988 ) ) ;
#60951=ORIENTED_EDGE ( 'NONE', *, *, #96058, .F. ) ;
#60952=ORIENTED_EDGE ( 'NONE', *, *, #44711, .F. ) ;
#60953=VERTEX_POINT ( 'NONE', #127202 ) ;
#60954=EDGE_CURVE ( 'NONE', #82935, #22615, #37531, .T. ) ;
#60955=PLANE ( 'NONE',  #111473 ) ;
#60956=EDGE_CURVE ( 'NONE', #100324, #82878, #107550, .T. ) ;
#60957=EDGE_CURVE ( 'NONE', #29934, #45445, #116255, .T. ) ;
#60959=CARTESIAN_POINT ( 'NONE',  ( 16.55874544816229132, -0.4845305829427751232, 6.091953208798936537 ) ) ;
#60960=AXIS2_PLACEMENT_3D ( 'NONE', #48240, #18772, #26030 ) ;
#60961=FACE_OUTER_BOUND ( 'NONE', #76429, .T. ) ;
#60962=AXIS2_PLACEMENT_3D ( 'NONE', #35033, #55931, #84756 ) ;
#60963=ADVANCED_FACE ( 'NONE', ( #78091 ), #57784, .T. ) ;
#60964=ADVANCED_FACE ( 'NONE', ( #70202 ), #31568, .T. ) ;
#60965=EDGE_LOOP ( 'NONE', ( #57529, #112712, #85799, #70417 ) ) ;
#60966=DIRECTION ( 'NONE',  ( -0.000000000000000000, -1.000000000000000000, -0.000000000000000000 ) ) ;
#60967=DIRECTION ( 'NONE',  ( -0.000000000000000000, 1.000000000000000000, -0.000000000000000000 ) ) ;
#60968=DIRECTION ( 'NONE',  ( 0.000000000000000000, 0.000000000000000000, -1.000000000000000000 ) ) ;
#60969=CARTESIAN_POINT ( 'NONE',  ( -12.09999999999999609, 2.500000000000000000, 0.7928203230275536750 ) ) ;
#60970=AXIS2_PLACEMENT_3D ( 'NONE', #121032, #43145, #122972 ) ;
#60971=EDGE_CURVE ( 'NONE', #64242, #98726, #110124, .T. ) ;
#60972=EDGE_CURVE ( 'NONE', #32336, #49835, #84958, .T. ) ;
#60973=DIRECTION ( 'NONE',  ( 0.000000000000000000, 0.000000000000000000, 1.000000000000000000 ) ) ;
#60974=CONICAL_SURFACE ( 'NONE', #4508, 0.09999999999999982514, 0.003490658503988666988 ) ;
#60975=ORIENTED_EDGE ( 'NONE', *, *, #64067, .F. ) ;
#60976=CARTESIAN_POINT ( 'NONE',  ( 32.28091694169009429, 1.401435235935458268, -4.680151435985021813 ) ) ;
#60977=PLANE ( 'NONE',  #49858 ) ;
#60978=EDGE_CURVE ( 'NONE', #62648, #123389, #18053, .T. ) ;
#60979=FACE_OUTER_BOUND ( 'NONE', #57377, .T. ) ;
#60980=AXIS2_PLACEMENT_3D ( 'NONE', #35712, #25224, #65140 ) ;
#60981=AXIS2_PLACEMENT_3D ( 'NONE', #4151, #25099, #103679 ) ;
#60982=CARTESIAN_POINT ( 'NONE',  ( -4.800000000000022915, 2.500000000000000000, 3.883716857408420431 ) ) ;
#60983=VERTEX_POINT ( 'NONE', #60403 ) ;
#60984=AXIS2_PLACEMENT_3D ( 'NONE', #66435, #95903, #124069 ) ;
#60985=VERTEX_POINT ( 'NONE', #51223 ) ;
#60987=DIRECTION ( 'NONE',  ( -4.274815082592931898E-19, -0.9999939076577903929, -0.003490651415223739937 ) ) ;
#60988=AXIS2_PLACEMENT_3D ( 'NONE', #117469, #129291, #119424 ) ;
#60989=LINE ( 'NONE', #22378, #28893 ) ;
#60990=EDGE_LOOP ( 'NONE', ( #109978, #30944, #110629, #40931 ) ) ;
#60991=PLANE ( 'NONE',  #107511 ) ;
#60992=DIRECTION ( 'NONE',  ( 0.000000000000000000, -0.000000000000000000, 1.000000000000000000 ) ) ;
#60993=AXIS2_PLACEMENT_3D ( 'NONE', #62953, #31569, #81940 ) ;
#60994=AXIS2_PLACEMENT_3D ( 'NONE', #90710, #59343, #50788 ) ;
#60995=ORIENTED_EDGE ( 'NONE', *, *, #23953, .T. ) ;
#60996=DIRECTION ( 'NONE',  ( -0.000000000000000000, -1.000000000000000000, -0.000000000000000000 ) ) ;
#60997=EDGE_LOOP ( 'NONE', ( #7362, #52371 ) ) ;
#60998=DIRECTION ( 'NONE',  ( 0.000000000000000000, 1.000000000000000000, 0.000000000000000000 ) ) ;
#60999=ORIENTED_EDGE ( 'NONE', *, *, #119490, .T. ) ;
#61000=ORIENTED_EDGE ( 'NONE', *, *, #38145, .F. ) ;
#61001=CARTESIAN_POINT ( 'NONE',  ( 5.849999999999931255, 12.50000000000000000, 2.857883832488649301 ) ) ;
#61002=CARTESIAN_POINT ( 'NONE',  ( -0.8500000000000382805, 12.50000000000000000, -5.867463478539787225 ) ) ;
#61003=ORIENTED_EDGE ( 'NONE', *, *, #60365, .T. ) ;
#61004=EDGE_LOOP ( 'NONE', ( #11029, #82921, #27573, #123773 ) ) ;
#61005=CARTESIAN_POINT ( 'NONE',  ( -8.100000000000010303, 12.50000000000000000, 3.983716857408420964 ) ) ;
#61006=CARTESIAN_POINT ( 'NONE',  ( 1.449999999999951328, 2.500000000000000000, -1.818653347947326138 ) ) ;
#61007=ORIENTED_EDGE ( 'NONE', *, *, #21054, .F. ) ;
#61008=DIRECTION ( 'NONE',  ( 0.000000000000000000, 0.000000000000000000, 1.000000000000000000 ) ) ;
#61010=EDGE_CURVE ( 'NONE', #124302, #43675, #112062, .T. ) ;
#61011=DIRECTION ( 'NONE',  ( -0.000000000000000000, 1.000000000000000000, -0.000000000000000000 ) ) ;
#61012=AXIS2_PLACEMENT_3D ( 'NONE', #117152, #107357, #57626 ) ;
#61013=DIRECTION ( 'NONE',  ( -0.000000000000000000, -1.000000000000000000, -0.000000000000000000 ) ) ;
#61014=FACE_OUTER_BOUND ( 'NONE', #38553, .T. ) ;
#61015=AXIS2_PLACEMENT_3D ( 'NONE', #89443, #20071, #108429 ) ;
#61016=AXIS2_PLACEMENT_3D ( 'NONE', #52553, #80086, #122590 ) ;
#61017=CARTESIAN_POINT ( 'NONE',  ( -6.050000000000020250, 12.50000000000000000, -6.906693963081115939 ) ) ;
#61018=DIRECTION ( 'NONE',  ( -0.000000000000000000, 1.000000000000000000, -0.000000000000000000 ) ) ;
#61019=CONICAL_SURFACE ( 'NONE', #67344, 0.1000000000000002554, 0.003490658503988666988 ) ;
#61020=ORIENTED_EDGE ( 'NONE', *, *, #110402, .F. ) ;
#61021=CIRCLE ( 'NONE', #121661, 0.1000000000000002554 ) ;
#61022=EDGE_LOOP ( 'NONE', ( #82178, #56291 ) ) ;
#61023=CARTESIAN_POINT ( 'NONE',  ( -10.85000000000000142, 12.50000000000000000, -2.099970236277060476 ) ) ;
#61025=LINE ( 'NONE', #49948, #18303 ) ;
#61026=CARTESIAN_POINT ( 'NONE',  ( 15.59999999999988951, 2.500000000000000000, -0.2464101615137783419 ) ) ;
#61027=AXIS2_PLACEMENT_3D ( 'NONE', #91961, #50750, #42893 ) ;
#61028=CARTESIAN_POINT ( 'NONE',  ( 5.599999999999931255, 12.50000000000000000, 4.676537180435972552 ) ) ;
#61029=ORIENTED_EDGE ( 'NONE', *, *, #22219, .F. ) ;
#61030=VERTEX_POINT ( 'NONE', #11270 ) ;
#61031=FACE_BOUND ( 'NONE', #42886, .T. ) ;
#61032=ORIENTED_EDGE ( 'NONE', *, *, #117850, .T. ) ;
#61033=DIRECTION ( 'NONE',  ( -0.000000000000000000, -1.000000000000000000, -0.000000000000000000 ) ) ;
#61035=VECTOR ( 'NONE', #105122, 1000.000000000000000 ) ;
#61036=DIRECTION ( 'NONE',  ( -0.000000000000000000, 1.000000000000000000, -0.000000000000000000 ) ) ;
#61037=DIRECTION ( 'NONE',  ( 0.000000000000000000, 1.000000000000000000, 0.000000000000000000 ) ) ;
#61038=DIRECTION ( 'NONE',  ( 0.000000000000000000, -0.000000000000000000, 1.000000000000000000 ) ) ;
#61039=DIRECTION ( 'NONE',  ( 0.000000000000000000, 1.000000000000000000, 0.000000000000000000 ) ) ;
#61040=DIRECTION ( 'NONE',  ( 0.000000000000000000, 0.000000000000000000, 1.000000000000000000 ) ) ;
#61041=DIRECTION ( 'NONE',  ( -0.000000000000000000, -1.000000000000000000, -0.000000000000000000 ) ) ;
#61042=DIRECTION ( 'NONE',  ( 0.000000000000000000, -0.000000000000000000, 1.000000000000000000 ) ) ;
#61043=DIRECTION ( 'NONE',  ( 0.000000000000000000, 1.000000000000000000, 0.000000000000000000 ) ) ;
#61044=CARTESIAN_POINT ( 'NONE',  ( -10.85000000000000142, 2.500000000000000000, 6.495190528383297135 ) ) ;
#61045=VERTEX_POINT ( 'NONE', #13189 ) ;
#61046=EDGE_LOOP ( 'NONE', ( #4719, #105219, #29637, #8248 ) ) ;
#61047=ORIENTED_EDGE ( 'NONE', *, *, #90134, .T. ) ;
#61048=ORIENTED_EDGE ( 'NONE', *, *, #51155, .F. ) ;
#61049=DIRECTION ( 'NONE',  ( -0.000000000000000000, -1.000000000000000000, -0.000000000000000000 ) ) ;
#61050=DIRECTION ( 'NONE',  ( 0.000000000000000000, 1.000000000000000000, 0.000000000000000000 ) ) ;
#61051=ORIENTED_EDGE ( 'NONE', *, *, #71100, .F. ) ;
#61052=VERTEX_POINT ( 'NONE', #61017 ) ;
#61053=ORIENTED_EDGE ( 'NONE', *, *, #122145, .T. ) ;
#61054=DIRECTION ( 'NONE',  ( 0.000000000000000000, 0.000000000000000000, 1.000000000000000000 ) ) ;
#61055=VECTOR ( 'NONE', #20717, 1000.000000000000000 ) ;
#61056=AXIS2_PLACEMENT_3D ( 'NONE', #77363, #14554, #55147 ) ;
#61057=EDGE_CURVE ( 'NONE', #52824, #29223, #89832, .T. ) ;
#61058=LINE ( 'NONE', #9394, #57196 ) ;
#61059=DIRECTION ( 'NONE',  ( -4.274815082592931898E-19, -0.9999939076577903929, -0.003490651415223739937 ) ) ;
#61060=FACE_OUTER_BOUND ( 'NONE', #85956, .T. ) ;
#61061=DIRECTION ( 'NONE',  ( 0.000000000000000000, -0.9999939076577903929, 0.003490651415223739937 ) ) ;
#61062=DIRECTION ( 'NONE',  ( 0.000000000000000000, 0.000000000000000000, -1.000000000000000000 ) ) ;
#61063=LINE ( 'NONE', #102291, #49624 ) ;
#61064=EDGE_CURVE ( 'NONE', #73869, #58451, #30607, .T. ) ;
#61065=VERTEX_POINT ( 'NONE', #21751 ) ;
#61067=EDGE_CURVE ( 'NONE', #37903, #1292, #7590, .T. ) ;
#61068=VECTOR ( 'NONE', #50775, 1000.000000000000000 ) ;
#61069=CARTESIAN_POINT ( 'NONE',  ( 5.199999999999937117, 12.50000000000000000, -4.611443907251940644 ) ) ;
#61070=EDGE_LOOP ( 'NONE', ( #70572, #98464, #83721, #48150 ) ) ;
#61071=CIRCLE ( 'NONE', #121701, 0.06509327318403745899 ) ;
#61072=ORIENTED_EDGE ( 'NONE', *, *, #90042, .F. ) ;
#61073=CIRCLE ( 'NONE', #59020, 0.06509327318403745899 ) ;
#61074=ORIENTED_EDGE ( 'NONE', *, *, #1850, .F. ) ;
#61075=EDGE_CURVE ( 'NONE', #30951, #110642, #61685, .T. ) ;
#61076=CARTESIAN_POINT ( 'NONE',  ( -7.300000000000016698, 12.50000000000000000, -0.4115034346978157509 ) ) ;
#61077=ADVANCED_FACE ( 'NONE', ( #40102 ), #15991, .T. ) ;
#61078=EDGE_CURVE ( 'NONE', #101182, #48101, #42702, .T. ) ;
#61079=ORIENTED_EDGE ( 'NONE', *, *, #15550, .T. ) ;
#61080=ORIENTED_EDGE ( 'NONE', *, *, #78394, .T. ) ;
#61081=ADVANCED_FACE ( 'NONE', ( #92407 ), #21091, .T. ) ;
#61082=EDGE_CURVE ( 'NONE', #15541, #126358, #82611, .T. ) ;
#61083=VERTEX_POINT ( 'NONE', #90464 ) ;
#61084=AXIS2_PLACEMENT_3D ( 'NONE', #75950, #76609, #87704 ) ;
#61085=CARTESIAN_POINT ( 'NONE',  ( -5.850000000000018296, 2.500000000000000000, 5.802370205355744659 ) ) ;
#61087=DIRECTION ( 'NONE',  ( -0.000000000000000000, 1.000000000000000000, -0.000000000000000000 ) ) ;
#61088=FACE_OUTER_BOUND ( 'NONE', #30101, .T. ) ;
#61089=CIRCLE ( 'NONE', #40168, 0.06509327318403745899 ) ;
#61090=CARTESIAN_POINT ( 'NONE',  ( -4.600000000000024514, 2.500000000000000000, 3.737306695894644371 ) ) ;
#61091=CARTESIAN_POINT ( 'NONE',  ( -8.750000000000005329, 2.500000000000000000, 5.702370205355745014 ) ) ;
#61092=ADVANCED_FACE ( 'NONE', ( #72142 ), #105805, .T. ) ;
#61093=AXIS2_PLACEMENT_3D ( 'NONE', #119131, #20283, #49117 ) ;
#61094=DIRECTION ( 'NONE',  ( 0.000000000000000000, 0.000000000000000000, 1.000000000000000000 ) ) ;
#61095=VERTEX_POINT ( 'NONE', #12551 ) ;
#61096=CARTESIAN_POINT ( 'NONE',  ( 9.399999999999915090, 12.50000000000000000, 4.676537180435972552 ) ) ;
#61098=CARTESIAN_POINT ( 'NONE',  ( 7.899999999999924860, 12.50000000000000000, 3.702399969078682407 ) ) ;
#61099=DIRECTION ( 'NONE',  ( 0.000000000000000000, 0.000000000000000000, 1.000000000000000000 ) ) ;
#61100=ORIENTED_EDGE ( 'NONE', *, *, #58085, .F. ) ;
#61101=CARTESIAN_POINT ( 'NONE',  ( 5.599999999999933031, 12.50000000000000000, 0.3464101615137735735 ) ) ;
#61102=LINE ( 'NONE', #50017, #118904 ) ;
#61103=ORIENTED_EDGE ( 'NONE', *, *, #111890, .T. ) ;
#61104=CARTESIAN_POINT ( 'NONE',  ( 9.999999999999952038, 12.50000000000000000, 0.06509327318403515528 ) ) ;
#61105=ORIENTED_EDGE ( 'NONE', *, *, #55192, .F. ) ;
#61106=ORIENTED_EDGE ( 'NONE', *, *, #67577, .T. ) ;
#61107=DIRECTION ( 'NONE',  ( 0.000000000000000000, 0.000000000000000000, 1.000000000000000000 ) ) ;
#61108=CARTESIAN_POINT ( 'NONE',  ( 3.949999999999942446, 2.500000000000000000, -6.741600689897078169 ) ) ;
#61109=CARTESIAN_POINT ( 'NONE',  ( -11.24999999999996270, 2.500000000000000000, 2.265063509461097357 ) ) ;
#61110=CARTESIAN_POINT ( 'NONE',  ( -2.300000000000033573, 2.500000000000000000, 4.776537180435972196 ) ) ;
#61111=FACE_OUTER_BOUND ( 'NONE', #11638, .T. ) ;
#61112=ORIENTED_EDGE ( 'NONE', *, *, #18717, .F. ) ;
#61113=DIRECTION ( 'NONE',  ( -0.000000000000000000, 1.000000000000000000, -0.000000000000000000 ) ) ;
#61114=VECTOR ( 'NONE', #127983, 1000.000000000000000 ) ;
#61115=CIRCLE ( 'NONE', #50652, 0.06509327318403745899 ) ;
#61116=AXIS2_PLACEMENT_3D ( 'NONE', #41311, #30847, #30204 ) ;
#61117=EDGE_CURVE ( 'NONE', #109003, #79439, #118409, .T. ) ;
#61118=EDGE_CURVE ( 'NONE', #1292, #37903, #26396, .T. ) ;
#61119=ORIENTED_EDGE ( 'NONE', *, *, #75003, .F. ) ;
#61120=DIRECTION ( 'NONE',  ( 0.000000000000000000, -0.000000000000000000, 1.000000000000000000 ) ) ;
#61121=LINE ( 'NONE', #69000, #70998 ) ;
#61122=AXIS2_PLACEMENT_3D ( 'NONE', #71370, #1996, #21653 ) ;
#61123=AXIS2_PLACEMENT_3D ( 'NONE', #4419, #63379, #81093 ) ;
#61125=AXIS2_PLACEMENT_3D ( 'NONE', #102125, #113881, #94228 ) ;
#61126=AXIS2_PLACEMENT_3D ( 'NONE', #106918, #17234, #89863 ) ;
#61127=AXIS2_PLACEMENT_3D ( 'NONE', #30021, #87623, #120325 ) ;
#61130=DIRECTION ( 'NONE',  ( 0.000000000000000000, 0.000000000000000000, 1.000000000000000000 ) ) ;
#61131=ADVANCED_FACE ( 'NONE', ( #113336 ), #9657, .T. ) ;
#61132=FACE_OUTER_BOUND ( 'NONE', #21094, .T. ) ;
#61133=DIRECTION ( 'NONE',  ( -0.000000000000000000, -1.000000000000000000, -0.000000000000000000 ) ) ;
#61134=ORIENTED_EDGE ( 'NONE', *, *, #26180, .F. ) ;
#61135=AXIS2_PLACEMENT_3D ( 'NONE', #90878, #71232, #31976 ) ;
#61136=ADVANCED_FACE ( 'NONE', ( #114622 ), #93075, .T. ) ;
#61137=CARTESIAN_POINT ( 'NONE',  ( -8.750000000000010658, 12.50000000000000000, 2.857883832488649301 ) ) ;
#61138=ADVANCED_FACE ( 'NONE', ( #24319 ), #17545, .T. ) ;
#61139=DIRECTION ( 'NONE',  ( 0.000000000000000000, 0.000000000000000000, 1.000000000000000000 ) ) ;
#61140=DIRECTION ( 'NONE',  ( 0.000000000000000000, 1.000000000000000000, 0.000000000000000000 ) ) ;
#61141=ORIENTED_EDGE ( 'NONE', *, *, #63441, .T. ) ;
#61142=EDGE_CURVE ( 'NONE', #50060, #84067, #51620, .T. ) ;
#61143=DIRECTION ( 'NONE',  ( -0.000000000000000000, 1.000000000000000000, -0.000000000000000000 ) ) ;
#61144=AXIS2_PLACEMENT_3D ( 'NONE', #90755, #10883, #9620 ) ;
#61145=ORIENTED_EDGE ( 'NONE', *, *, #84843, .F. ) ;
#61146=ORIENTED_EDGE ( 'NONE', *, *, #15949, .T. ) ;
#61147=FACE_OUTER_BOUND ( 'NONE', #91047, .T. ) ;
#61148=ORIENTED_EDGE ( 'NONE', *, *, #75952, .F. ) ;
#61149=CARTESIAN_POINT ( 'NONE',  ( 15.05551045035344870, -2.483581587658457490, -4.666934263344250766 ) ) ;
#61150=DIRECTION ( 'NONE',  ( 0.000000000000000000, 0.000000000000000000, 1.000000000000000000 ) ) ;
#61151=DIRECTION ( 'NONE',  ( 0.000000000000000000, 0.000000000000000000, 1.000000000000000000 ) ) ;
#61152=CIRCLE ( 'NONE', #98790, 0.06509327318403745899 ) ;
#61153=ORIENTED_EDGE ( 'NONE', *, *, #52347, .F. ) ;
#61154=AXIS2_PLACEMENT_3D ( 'NONE', #82617, #12556, #103541 ) ;
#61155=CARTESIAN_POINT ( 'NONE',  ( 3.949999999999942446, 12.50000000000000000, -2.511473670974877948 ) ) ;
#61156=CARTESIAN_POINT ( 'NONE',  ( 4.349999999999936584, 2.500000000000000000, 6.248780366869520542 ) ) ;
#61157=CARTESIAN_POINT ( 'NONE',  ( 17.46754056294898660, -1.506946016785628562, -5.249106941592948772 ) ) ;
#61159=CONICAL_SURFACE ( 'NONE', #84129, 0.1000000000000002554, 0.003490658503988666988 ) ;
#61160=ORIENTED_EDGE ( 'NONE', *, *, #5116, .T. ) ;
#61161=CONICAL_SURFACE ( 'NONE', #36029, 0.1000000000000000472, 0.003490658503988666988 ) ;
#61162=AXIS2_PLACEMENT_3D ( 'NONE', #53169, #34833, #83274 ) ;
#61163=ORIENTED_EDGE ( 'NONE', *, *, #82555, .T. ) ;
#61164=ORIENTED_EDGE ( 'NONE', *, *, #60312, .T. ) ;
#61165=CARTESIAN_POINT ( 'NONE',  ( 14.59999999999989484, 2.500000000000000000, -0.7928203230275542301 ) ) ;
#61166=DIRECTION ( 'NONE',  ( 0.000000000000000000, -0.000000000000000000, 1.000000000000000000 ) ) ;
#61167=DIRECTION ( 'NONE',  ( -0.000000000000000000, 1.000000000000000000, -0.000000000000000000 ) ) ;
#61168=FACE_BOUND ( 'NONE', #109230, .T. ) ;
#61169=VERTEX_POINT ( 'NONE', #24961 ) ;
#61170=LINE ( 'NONE', #42179, #71841 ) ;
#61171=LINE ( 'NONE', #101093, #75322 ) ;
#61172=AXIS2_PLACEMENT_3D ( 'NONE', #40580, #80495, #110578 ) ;
#61173=ORIENTED_EDGE ( 'NONE', *, *, #83091, .T. ) ;
#61174=DIRECTION ( 'NONE',  ( -0.000000000000000000, -1.000000000000000000, -0.000000000000000000 ) ) ;
#61175=PLANE ( 'NONE',  #45014 ) ;
#61176=EDGE_CURVE ( 'NONE', #52125, #58340, #13940, .T. ) ;
#61177=CONICAL_SURFACE ( 'NONE', #90402, 0.1000000000000000056, 0.003490658503988666988 ) ;
#61178=CIRCLE ( 'NONE', #8834, 0.1000000000000002554 ) ;
#61179=VECTOR ( 'NONE', #123043, 1000.000000000000000 ) ;
#61180=DIRECTION ( 'NONE',  ( 0.000000000000000000, 0.000000000000000000, -1.000000000000000000 ) ) ;
#61181=PLANE ( 'NONE',  #103126 ) ;
#61182=DIRECTION ( 'NONE',  ( -0.000000000000000000, 1.000000000000000000, -0.000000000000000000 ) ) ;
#61183=DIRECTION ( 'NONE',  ( 0.000000000000000000, 0.000000000000000000, -1.000000000000000000 ) ) ;
#61184=AXIS2_PLACEMENT_3D ( 'NONE', #89513, #50882, #48302 ) ;
#61185=CARTESIAN_POINT ( 'NONE',  ( 1.699999999999951994, 2.500000000000000000, -4.330127018922201643 ) ) ;
#61186=ORIENTED_EDGE ( 'NONE', *, *, #65176, .F. ) ;
#61187=CIRCLE ( 'NONE', #86296, 0.1000000000000002554 ) ;
#61189=ORIENTED_EDGE ( 'NONE', *, *, #107948, .F. ) ;
#61190=ORIENTED_EDGE ( 'NONE', *, *, #5371, .T. ) ;
#61191=PLANE ( 'NONE',  #53725 ) ;
#61192=CARTESIAN_POINT ( 'NONE',  ( 0.8499999999999545697, 2.500000000000000000, 2.757883832488649656 ) ) ;
#61193=ORIENTED_EDGE ( 'NONE', *, *, #93707, .F. ) ;
#61194=EDGE_CURVE ( 'NONE', #49661, #41193, #24418, .T. ) ;
#61195=FACE_BOUND ( 'NONE', #18356, .T. ) ;
#61196=DIRECTION ( 'NONE',  ( 0.000000000000000000, -0.000000000000000000, 1.000000000000000000 ) ) ;
#61197=CARTESIAN_POINT ( 'NONE',  ( -4.200000000000029488, 2.500000000000000000, -4.430127018922202176 ) ) ;
#61199=DIRECTION ( 'NONE',  ( -0.000000000000000000, 1.000000000000000000, -0.000000000000000000 ) ) ;
#61200=DIRECTION ( 'NONE',  ( -0.000000000000000000, -1.000000000000000000, -0.000000000000000000 ) ) ;
#61201=DIRECTION ( 'NONE',  ( 0.000000000000000000, 0.000000000000000000, 1.000000000000000000 ) ) ;
#61202=DIRECTION ( 'NONE',  ( 0.000000000000000000, -0.000000000000000000, 1.000000000000000000 ) ) ;
#61203=DIRECTION ( 'NONE',  ( -0.000000000000000000, 1.000000000000000000, -0.000000000000000000 ) ) ;
#61204=AXIS2_PLACEMENT_3D ( 'NONE', #53067, #63535, #15036 ) ;
#61205=CARTESIAN_POINT ( 'NONE',  ( 7.499999999999927169, 2.500000000000000000, 3.537306695894645081 ) ) ;
#61206=ORIENTED_EDGE ( 'NONE', *, *, #20042, .F. ) ;
#61207=ORIENTED_EDGE ( 'NONE', *, *, #3988, .T. ) ;
#61208=ORIENTED_EDGE ( 'NONE', *, *, #47537, .T. ) ;
#61209=ORIENTED_EDGE ( 'NONE', *, *, #83512, .T. ) ;
#61210=ORIENTED_EDGE ( 'NONE', *, *, #118537, .F. ) ;
#61211=AXIS2_PLACEMENT_3D ( 'NONE', #10145, #59914, #88703 ) ;
#61212=ORIENTED_EDGE ( 'NONE', *, *, #31412, .F. ) ;
#61213=CONICAL_SURFACE ( 'NONE', #40288, 0.1000000000000002554, 0.003490658503988666988 ) ;
#61214=CIRCLE ( 'NONE', #59064, 0.06509327318403745899 ) ;
#61215=DIRECTION ( 'NONE',  ( -0.000000000000000000, -1.000000000000000000, -0.000000000000000000 ) ) ;
#61216=VERTEX_POINT ( 'NONE', #43970 ) ;
#61217=VECTOR ( 'NONE', #80579, 1000.000000000000000 ) ;
#61218=AXIS2_PLACEMENT_3D ( 'NONE', #87506, #128097, #79634 ) ;
#61219=VECTOR ( 'NONE', #74319, 1000.000000000000000 ) ;
#61220=ADVANCED_FACE ( 'NONE', ( #107225 ), #34906, .T. ) ;
#61221=CARTESIAN_POINT ( 'NONE',  ( 17.19804440726978001, 0.4677972980984275164, 5.492654682185340143 ) ) ;
#61222=CARTESIAN_POINT ( 'NONE',  ( 13.91976764310545356, -2.499999999999999556, 6.779443705068508130 ) ) ;
#61223=CARTESIAN_POINT ( 'NONE',  ( -4.150000000000027889, 2.500000000000000000, -6.395190528383301931 ) ) ;
#61224=CARTESIAN_POINT ( 'NONE',  ( -4.200000000000025935, 12.50000000000000000, -2.385244779468109755E-15 ) ) ;
#61225=VECTOR ( 'NONE', #55586, 1000.000000000000000 ) ;
#61226=VECTOR ( 'NONE', #93774, 1000.000000000000000 ) ;
#61227=AXIS2_PLACEMENT_3D ( 'NONE', #113706, #64598, #105163 ) ;
#61228=ORIENTED_EDGE ( 'NONE', *, *, #18074, .T. ) ;
#61229=CARTESIAN_POINT ( 'NONE',  ( 3.549999999999944755, 2.500000000000000000, -6.741600689897077281 ) ) ;
#61230=VERTEX_POINT ( 'NONE', #87578 ) ;
#61231=EDGE_LOOP ( 'NONE', ( #21846, #66706 ) ) ;
#61232=DIRECTION ( 'NONE',  ( 0.000000000000000000, 0.000000000000000000, -1.000000000000000000 ) ) ;
#61233=EDGE_CURVE ( 'NONE', #111264, #83483, #95528, .T. ) ;
#61234=DIRECTION ( 'NONE',  ( -4.274815082592931898E-19, -0.9999939076577903929, -0.003490651415223739937 ) ) ;
#61235=DIRECTION ( 'NONE',  ( 0.000000000000000000, 0.000000000000000000, 1.000000000000000000 ) ) ;
#61236=ADVANCED_FACE ( 'NONE', ( #47676 ), #83872, .T. ) ;
#61237=ADVANCED_FACE ( 'NONE', ( #28030 ), #64871, .T. ) ;
#61238=EDGE_CURVE ( 'NONE', #88434, #51372, #107870, .T. ) ;
#61239=ORIENTED_EDGE ( 'NONE', *, *, #98015, .F. ) ;
#61240=ORIENTED_EDGE ( 'NONE', *, *, #101024, .F. ) ;
#61241=AXIS2_PLACEMENT_3D ( 'NONE', #69677, #59888, #275 ) ;
#61242=DIRECTION ( 'NONE',  ( 0.000000000000000000, -0.000000000000000000, 1.000000000000000000 ) ) ;
#61243=DIRECTION ( 'NONE',  ( 0.000000000000000000, 0.000000000000000000, 1.000000000000000000 ) ) ;
#61244=EDGE_CURVE ( 'NONE', #21424, #120749, #124766, .T. ) ;
#61245=DIRECTION ( 'NONE',  ( 0.000000000000000000, -0.000000000000000000, 1.000000000000000000 ) ) ;
#61246=DIRECTION ( 'NONE',  ( -4.274815082592931898E-19, -0.9999939076577903929, -0.003490651415223739937 ) ) ;
#61247=VERTEX_POINT ( 'NONE', #34805 ) ;
#61248=CARTESIAN_POINT ( 'NONE',  ( -0.4000000000000392131, 12.50000000000000000, -4.330127018922201643 ) ) ;
#61249=ADVANCED_FACE ( 'NONE', ( #125095 ), #45363, .T. ) ;
#61250=AXIS2_PLACEMENT_3D ( 'NONE', #42810, #63712, #82721 ) ;
#61251=EDGE_LOOP ( 'NONE', ( #94209, #54483 ) ) ;
#61252=CARTESIAN_POINT ( 'NONE',  ( 8.340322510150738111, -2.500000000000000444, 8.517653998215580557 ) ) ;
#61253=CONICAL_SURFACE ( 'NONE', #120028, 0.09999999999999982514, 0.003490658503988666988 ) ;
#61254=ADVANCED_FACE ( 'NONE', ( #85168 ), #32843, .T. ) ;
#61255=AXIS2_PLACEMENT_3D ( 'NONE', #117180, #78603, #58313 ) ;
#61256=EDGE_CURVE ( 'NONE', #97131, #73152, #97567, .T. ) ;
#61257=ORIENTED_EDGE ( 'NONE', *, *, #123006, .T. ) ;
#61258=CARTESIAN_POINT ( 'NONE',  ( -6.249999999999981348, 12.50000000000000000, 2.230156782645134950 ) ) ;
#61259=DIRECTION ( 'NONE',  ( -0.000000000000000000, -1.000000000000000000, -0.000000000000000000 ) ) ;
#61260=DIRECTION ( 'NONE',  ( -4.274815082592931898E-19, -0.9999939076577903929, -0.003490651415223739937 ) ) ;
#61262=CARTESIAN_POINT ( 'NONE',  ( 0.5999999999999621192, 2.500000000000000000, 0.2464101615137758439 ) ) ;
#61263=AXIS2_PLACEMENT_3D ( 'NONE', #88344, #69358, #78570 ) ;
#61264=EDGE_CURVE ( 'NONE', #119243, #122680, #9751, .T. ) ;
#61265=VERTEX_POINT ( 'NONE', #89522 ) ;
#61266=AXIS2_PLACEMENT_3D ( 'NONE', #72166, #2763, #104189 ) ;
#61267=CARTESIAN_POINT ( 'NONE',  ( -2.700000000000030820, 2.500000000000000000, -3.983716857408426293 ) ) ;
#61268=FACE_OUTER_BOUND ( 'NONE', #76274, .T. ) ;
#61269=ORIENTED_EDGE ( 'NONE', *, *, #97287, .T. ) ;
#61270=EDGE_LOOP ( 'NONE', ( #39692, #28617, #14360, #97503 ) ) ;
#61271=ORIENTED_EDGE ( 'NONE', *, *, #45296, .F. ) ;
#61272=CARTESIAN_POINT ( 'NONE',  ( 17.50000000000000000, 0.9166666666666685170, 2.864912725862981624 ) ) ;
#61273=LINE ( 'NONE', #81550, #19822 ) ;
#61274=CARTESIAN_POINT ( 'NONE',  ( 17.79089025268834590, 2.511997385349132195, 2.795007471442508606 ) ) ;
#61275=AXIS2_PLACEMENT_3D ( 'NONE', #85624, #16851, #86910 ) ;
#61276=PLANE ( 'NONE',  #126412 ) ;
#61277=CARTESIAN_POINT ( 'NONE',  ( 8.949999999999919353, 12.50000000000000000, 2.576566944158910744 ) ) ;
#61278=DIRECTION ( 'NONE',  ( -0.000000000000000000, -1.000000000000000000, -0.000000000000000000 ) ) ;
#61279=CIRCLE ( 'NONE', #121909, 0.09999999999999982514 ) ;
#61280=DIRECTION ( 'NONE',  ( -0.000000000000000000, 1.000000000000000000, -0.000000000000000000 ) ) ;
#61281=CIRCLE ( 'NONE', #107231, 0.1000000000000000472 ) ;
#61282=CONICAL_SURFACE ( 'NONE', #21562, 0.09999999999999982514, 0.003490658503988666988 ) ;
#61283=FACE_OUTER_BOUND ( 'NONE', #10790, .T. ) ;
#61284=CONICAL_SURFACE ( 'NONE', #119758, 0.1000000000000002554, 0.003490658503988666988 ) ;
#61285=AXIS2_PLACEMENT_3D ( 'NONE', #4341, #44290, #84210 ) ;
#61286=EDGE_LOOP ( 'NONE', ( #43546, #30511, #17916, #11409 ) ) ;
#61288=CARTESIAN_POINT ( 'NONE',  ( 8.149999999999923972, 2.500000000000000000, 1.718653347947321386 ) ) ;
#61289=CARTESIAN_POINT ( 'NONE',  ( 7.049999999999928768, 2.500000000000000000, 6.395190528383296602 ) ) ;
#61290=DIRECTION ( 'NONE',  ( -0.000000000000000000, 1.000000000000000000, -0.000000000000000000 ) ) ;
#61291=ORIENTED_EDGE ( 'NONE', *, *, #105595, .T. ) ;
#61292=DIRECTION ( 'NONE',  ( 0.000000000000000000, 0.000000000000000000, -1.000000000000000000 ) ) ;
#61293=EDGE_CURVE ( 'NONE', #55263, #114720, #32763, .T. ) ;
#61294=ADVANCED_FACE ( 'NONE', ( #49620 ), #57882, .T. ) ;
#61295=DIRECTION ( 'NONE',  ( 0.000000000000000000, 1.000000000000000000, 0.000000000000000000 ) ) ;
#61296=DIRECTION ( 'NONE',  ( -4.274815082592931898E-19, -0.9999939076577903929, -0.003490651415223739937 ) ) ;
#61297=VERTEX_POINT ( 'NONE', #90812 ) ;
#61298=VECTOR ( 'NONE', #9731, 1000.000000000000000 ) ;
#61299=CONICAL_SURFACE ( 'NONE', #38315, 0.1000000000000000472, 0.003490658503988666988 ) ;
#61300=ORIENTED_EDGE ( 'NONE', *, *, #23768, .F. ) ;
#61301=EDGE_CURVE ( 'NONE', #5223, #103548, #28680, .T. ) ;
#61302=FACE_OUTER_BOUND ( 'NONE', #113323, .T. ) ;
#61303=VECTOR ( 'NONE', #52761, 1000.000000000000000 ) ;
#61304=EDGE_LOOP ( 'NONE', ( #127072, #97691, #15809, #46540 ) ) ;
#61305=CONICAL_SURFACE ( 'NONE', #113527, 0.1000000000000002554, 0.003490658503988666988 ) ;
#61306=ORIENTED_EDGE ( 'NONE', *, *, #3808, .T. ) ;
#61307=LINE ( 'NONE', #79645, #19735 ) ;
#61308=AXIS2_PLACEMENT_3D ( 'NONE', #50929, #111775, #81660 ) ;
#61309=CIRCLE ( 'NONE', #40387, 0.1000000000000002554 ) ;
#61310=DIRECTION ( 'NONE',  ( 0.000000000000000000, 0.000000000000000000, -1.000000000000000000 ) ) ;
#61311=CARTESIAN_POINT ( 'NONE',  ( 2.699999999999945555, 2.500000000000000000, 3.983716857408420076 ) ) ;
#61312=CARTESIAN_POINT ( 'NONE',  ( -6.850000000000017408, 2.500000000000000000, -6.048780366869526581 ) ) ;
#61313=CIRCLE ( 'NONE', #52905, 0.1000000000000000472 ) ;
#61314=ORIENTED_EDGE ( 'NONE', *, *, #69607, .T. ) ;
#61315=AXIS2_PLACEMENT_3D ( 'NONE', #50826, #72406, #73039 ) ;
#61316=VECTOR ( 'NONE', #102965, 1000.000000000000000 ) ;
#61317=DIRECTION ( 'NONE',  ( -0.000000000000000000, -1.000000000000000000, -0.000000000000000000 ) ) ;
#61318=ORIENTED_EDGE ( 'NONE', *, *, #5064, .F. ) ;
#61319=AXIS2_PLACEMENT_3D ( 'NONE', #125786, #4718, #123241 ) ;
#61321=DIRECTION ( 'NONE',  ( -0.000000000000000000, 1.000000000000000000, -0.000000000000000000 ) ) ;
#61322=AXIS2_PLACEMENT_3D ( 'NONE', #59690, #80599, #70136 ) ;
#61323=VERTEX_POINT ( 'NONE', #129481 ) ;
#61324=ORIENTED_EDGE ( 'NONE', *, *, #69680, .T. ) ;
#61325=EDGE_LOOP ( 'NONE', ( #43027, #11816, #76942, #4093 ) ) ;
#61326=ORIENTED_EDGE ( 'NONE', *, *, #69105, .F. ) ;
#61327=DIRECTION ( 'NONE',  ( 0.000000000000000000, -0.9999939076577903929, 0.003490651415223739937 ) ) ;
#61328=CARTESIAN_POINT ( 'NONE',  ( 7.314170287632372869, 1.499999999999873657, 9.688393442221709506 ) ) ;
#61329=DIRECTION ( 'NONE',  ( 0.000000000000000000, 0.000000000000000000, 1.000000000000000000 ) ) ;
#61330=FACE_BOUND ( 'NONE', #102523, .T. ) ;
#61331=DIRECTION ( 'NONE',  ( 0.000000000000000000, 0.000000000000000000, 1.000000000000000000 ) ) ;
#61333=CARTESIAN_POINT ( 'NONE',  ( 9.799999999999915445, 2.500000000000000000, -4.576537180435977348 ) ) ;
#61334=CARTESIAN_POINT ( 'NONE',  ( -3.550000000000031797, 2.500000000000000000, -6.148780366869526226 ) ) ;
#61335=FACE_OUTER_BOUND ( 'NONE', #16337, .T. ) ;
#61336=LINE ( 'NONE', #23324, #11244 ) ;
#61337=CARTESIAN_POINT ( 'NONE',  ( -14.79999999999998295, 2.500000000000000000, -0.2464101615137760659 ) ) ;
#61338=VECTOR ( 'NONE', #92194, 1000.000000000000000 ) ;
#61340=CIRCLE ( 'NONE', #53029, 0.1000000000000000472 ) ;
#61341=PLANE ( 'NONE',  #116304 ) ;
#61342=VERTEX_POINT ( 'NONE', #8371 ) ;
#61343=EDGE_LOOP ( 'NONE', ( #24414, #113397, #34387, #78163 ) ) ;
#61344=ORIENTED_EDGE ( 'NONE', *, *, #66420, .T. ) ;
#61345=ORIENTED_EDGE ( 'NONE', *, *, #37426, .T. ) ;
#61346=EDGE_CURVE ( 'NONE', #75618, #64042, #1421, .T. ) ;
#61347=ORIENTED_EDGE ( 'NONE', *, *, #1504, .T. ) ;
#61348=CARTESIAN_POINT ( 'NONE',  ( -1.050000000000037792, 2.500000000000000000, 1.818653347947321475 ) ) ;
#61349=DIRECTION ( 'NONE',  ( -4.274815082592931898E-19, -0.9999939076577903929, -0.003490651415223739937 ) ) ;
#61350=ORIENTED_EDGE ( 'NONE', *, *, #99809, .T. ) ;
#61351=ADVANCED_FACE ( 'NONE', ( #68587 ), #85049, .T. ) ;
#61352=FACE_BOUND ( 'NONE', #8081, .T. ) ;
#61353=CONICAL_SURFACE ( 'NONE', #111513, 0.1000000000000002554, 0.003490658503988666988 ) ;
#61354=VECTOR ( 'NONE', #4389, 1000.000000000000000 ) ;
#61355=DIRECTION ( 'NONE',  ( 0.000000000000000000, -0.000000000000000000, 1.000000000000000000 ) ) ;
#61356=CONICAL_SURFACE ( 'NONE', #50887, 0.1000000000000000056, 0.003490658503988666988 ) ;
#61357=VECTOR ( 'NONE', #124404, 1000.000000000000000 ) ;
#61358=ORIENTED_EDGE ( 'NONE', *, *, #85480, .F. ) ;
#61361=ADVANCED_FACE ( 'NONE', ( #20790 ), #105987, .T. ) ;
#61362=CARTESIAN_POINT ( 'NONE',  ( 97.50000000000000000, 0.000000000000000000, 0.000000000000000000 ) ) ;
#61363=DIRECTION ( 'NONE',  ( 0.000000000000000000, 1.000000000000000000, 0.000000000000000000 ) ) ;
#61364=AXIS2_PLACEMENT_3D ( 'NONE', #63945, #54121, #44293 ) ;
#61365=ORIENTED_EDGE ( 'NONE', *, *, #128478, .T. ) ;
#61366=DIRECTION ( 'NONE',  ( 0.000000000000000000, 1.000000000000000000, 0.000000000000000000 ) ) ;
#61367=CONICAL_SURFACE ( 'NONE', #2777, 0.1000000000000002554, 0.003490658503988666988 ) ;
#61368=EDGE_LOOP ( 'NONE', ( #19531, #107987, #15825, #100583 ) ) ;
#61370=LINE ( 'NONE', #71836, #52876 ) ;
#61371=FACE_OUTER_BOUND ( 'NONE', #105884, .T. ) ;
#61372=VECTOR ( 'NONE', #83419, 1000.000000000000000 ) ;
#61373=VERTEX_POINT ( 'NONE', #479 ) ;
#61374=CARTESIAN_POINT ( 'NONE',  ( 6.049999999999934097, 12.50000000000000000, -2.511473670974877948 ) ) ;
#61375=CIRCLE ( 'NONE', #126209, 0.09999999999999982514 ) ;
#61376=DIRECTION ( 'NONE',  ( 0.7336674352945127264, 0.000000000000000000, -0.6795087154616723524 ) ) ;
#61377=CARTESIAN_POINT ( 'NONE',  ( -14.99999999999998224, 2.500000000000000000, -0.5928203230275518321 ) ) ;
#61378=EDGE_CURVE ( 'NONE', #101827, #128672, #126824, .T. ) ;
#61379=DIRECTION ( 'NONE',  ( 0.000000000000000000, -0.9999939076577903929, 0.003490651415223739937 ) ) ;
#61380=CARTESIAN_POINT ( 'NONE',  ( -12.89999999999999147, 2.500000000000000000, 4.922947341949748257 ) ) ;
#61381=VERTEX_POINT ( 'NONE', #120915 ) ;
#61382=DIRECTION ( 'NONE',  ( -0.000000000000000000, -1.000000000000000000, -0.000000000000000000 ) ) ;
#61383=ORIENTED_EDGE ( 'NONE', *, *, #91357, .T. ) ;
#61384=DIRECTION ( 'NONE',  ( 0.000000000000000000, 0.000000000000000000, 1.000000000000000000 ) ) ;
#61385=EDGE_CURVE ( 'NONE', #63267, #32002, #91318, .T. ) ;
#61386=ORIENTED_EDGE ( 'NONE', *, *, #27105, .F. ) ;
#61387=DIRECTION ( 'NONE',  ( -4.274815082592931898E-19, -0.9999939076577903929, -0.003490651415223739937 ) ) ;
#61388=ORIENTED_EDGE ( 'NONE', *, *, #108109, .F. ) ;
#61389=DIRECTION ( 'NONE',  ( -4.274815082592931898E-19, -0.9999939076577903929, -0.003490651415223739937 ) ) ;
#61390=CARTESIAN_POINT ( 'NONE',  ( -11.84999999999999787, 12.50000000000000000, -6.841600689897074261 ) ) ;
#61391=AXIS2_PLACEMENT_3D ( 'NONE', #50302, #128227, #88263 ) ;
#61392=ADVANCED_FACE ( 'NONE', ( #29974 ), #105894, .T. ) ;
#61393=PLANE ( 'NONE',  #63420 ) ;
#61394=CONICAL_SURFACE ( 'NONE', #21684, 0.1000000000000002554, 0.003490658503988666988 ) ;
#61395=DIRECTION ( 'NONE',  ( 0.000000000000000000, 1.000000000000000000, 0.000000000000000000 ) ) ;
#61396=EDGE_CURVE ( 'NONE', #36746, #117447, #101794, .T. ) ;
#61397=ADVANCED_FACE ( 'NONE', ( #20147 ), #80363, .T. ) ;
#61398=CARTESIAN_POINT ( 'NONE',  ( 16.73738517756865107, 0.6985710795863369071, -5.899868569652234385 ) ) ;
#61399=ADVANCED_FACE ( 'NONE', ( #10933 ), #5612, .T. ) ;
#61400=EDGE_LOOP ( 'NONE', ( #99452, #35046 ) ) ;
#61401=ORIENTED_EDGE ( 'NONE', *, *, #65626, .F. ) ;
#61402=EDGE_LOOP ( 'NONE', ( #84609, #22701, #38388, #39812 ) ) ;
#61403=FACE_OUTER_BOUND ( 'NONE', #23637, .T. ) ;
#61404=CONICAL_SURFACE ( 'NONE', #11203, 0.09999999999999982514, 0.003490658503988666988 ) ;
#61405=AXIS2_PLACEMENT_3D ( 'NONE', #9905, #128419, #89111 ) ;
#61406=CONICAL_SURFACE ( 'NONE', #103151, 0.1000000000000002554, 0.003490658503988666988 ) ;
#61407=CARTESIAN_POINT ( 'NONE',  ( -3.469446951953614189E-14, 2.500000000000000000, -0.6928203230275519209 ) ) ;
#61408=CIRCLE ( 'NONE', #101098, 0.1000000000000000056 ) ;
#61409=EDGE_CURVE ( 'NONE', #84837, #129184, #79076, .T. ) ;
#61410=CONICAL_SURFACE ( 'NONE', #4932, 0.09999999999999982514, 0.003490658503988666988 ) ;
#61411=CARTESIAN_POINT ( 'NONE',  ( 12.89999999999990266, 2.500000000000000000, 3.637306695894644726 ) ) ;
#61412=ORIENTED_EDGE ( 'NONE', *, *, #9547, .F. ) ;
#61413=VERTEX_POINT ( 'NONE', #50253 ) ;
#61414=VERTEX_POINT ( 'NONE', #90145 ) ;
#61415=EDGE_CURVE ( 'NONE', #87657, #107252, #78819, .T. ) ;
#61416=CARTESIAN_POINT ( 'NONE',  ( -8.350000000000013856, 12.50000000000000000, -6.430097255199259010 ) ) ;
#61417=ORIENTED_EDGE ( 'NONE', *, *, #35989, .F. ) ;
#61418=CARTESIAN_POINT ( 'NONE',  ( -5.400000000000019895, 2.500000000000000000, 4.230127018922196669 ) ) ;
#61419=FACE_OUTER_BOUND ( 'NONE', #126601, .T. ) ;
#61420=CONICAL_SURFACE ( 'NONE', #25802, 0.1000000000000002554, 0.003490658503988666988 ) ;
#61421=EDGE_CURVE ( 'NONE', #81575, #7967, #3490, .T. ) ;
#61422=CIRCLE ( 'NONE', #128315, 0.1000000000000002554 ) ;
#61423=ADVANCED_FACE ( 'NONE', ( #122855 ), #93375, .T. ) ;
#61424=DIRECTION ( 'NONE',  ( 0.000000000000000000, 0.000000000000000000, 1.000000000000000000 ) ) ;
#61425=CARTESIAN_POINT ( 'NONE',  ( 8.149999999999920419, 2.500000000000000000, 6.841600689897072485 ) ) ;
#61426=DIRECTION ( 'NONE',  ( -0.000000000000000000, -1.000000000000000000, -0.000000000000000000 ) ) ;
#61427=DIRECTION ( 'NONE',  ( -0.000000000000000000, -1.000000000000000000, -0.000000000000000000 ) ) ;
#61428=LINE ( 'NONE', #84255, #78117 ) ;
#61429=AXIS2_PLACEMENT_3D ( 'NONE', #125008, #124373, #83790 ) ;
#61430=CARTESIAN_POINT ( 'NONE',  ( 7.499999999999927169, 12.50000000000000000, -5.022947341949754119 ) ) ;
#61431=EDGE_CURVE ( 'NONE', #102257, #18238, #20219, .T. ) ;
#61432=ORIENTED_EDGE ( 'NONE', *, *, #58462, .T. ) ;
#61433=DIRECTION ( 'NONE',  ( 0.000000000000000000, -0.000000000000000000, 1.000000000000000000 ) ) ;
#61434=CARTESIAN_POINT ( 'NONE',  ( -12.09999999999999432, 12.50000000000000000, 5.022947341949748790 ) ) ;
#61435=ORIENTED_EDGE ( 'NONE', *, *, #6979, .F. ) ;
#61436=ORIENTED_EDGE ( 'NONE', *, *, #90614, .T. ) ;
#61438=DIRECTION ( 'NONE',  ( 0.000000000000000000, 1.000000000000000000, 0.000000000000000000 ) ) ;
#61439=CARTESIAN_POINT ( 'NONE',  ( -8.350000000000013856, 12.50000000000000000, -2.165063509461101710 ) ) ;
#61440=CIRCLE ( 'NONE', #48910, 0.06509327318403745899 ) ;
#61441=DIRECTION ( 'NONE',  ( 0.000000000000000000, 1.000000000000000000, 0.000000000000000000 ) ) ;
#61442=CARTESIAN_POINT ( 'NONE',  ( -15.19999999999998153, 12.50000000000000000, -0.2813168883297385570 ) ) ;
#61443=CARTESIAN_POINT ( 'NONE',  ( -3.150000000000030109, 12.50000000000000000, 1.818653347947321475 ) ) ;
#61444=DIRECTION ( 'NONE',  ( 0.000000000000000000, 0.000000000000000000, 1.000000000000000000 ) ) ;
#61445=DIRECTION ( 'NONE',  ( 0.000000000000000000, 1.000000000000000000, 0.000000000000000000 ) ) ;
#61446=AXIS2_PLACEMENT_3D ( 'NONE', #49563, #121488, #39754 ) ;
#61447=CARTESIAN_POINT ( 'NONE',  ( -11.04999999999999893, 2.500000000000000000, 6.048780366869520364 ) ) ;
#61448=CIRCLE ( 'NONE', #88618, 0.1000000000000002554 ) ;
#61449=ORIENTED_EDGE ( 'NONE', *, *, #54609, .F. ) ;
#61450=AXIS2_PLACEMENT_3D ( 'NONE', #23647, #103504, #22380 ) ;
#61451=EDGE_LOOP ( 'NONE', ( #113823, #42038 ) ) ;
#61452=ORIENTED_EDGE ( 'NONE', *, *, #54143, .T. ) ;
#61453=VERTEX_POINT ( 'NONE', #93395 ) ;
#61454=AXIS2_PLACEMENT_3D ( 'NONE', #26720, #124920, #75173 ) ;
#61455=DIRECTION ( 'NONE',  ( 0.000000000000000000, 0.000000000000000000, -1.000000000000000000 ) ) ;
#61456=CARTESIAN_POINT ( 'NONE',  ( -11.24999999999999822, 2.500000000000000000, 1.472243186433545459 ) ) ;
#61457=AXIS2_PLACEMENT_3D ( 'NONE', #38415, #69131, #68490 ) ;
#61458=ORIENTED_EDGE ( 'NONE', *, *, #99203, .T. ) ;
#61459=FACE_OUTER_BOUND ( 'NONE', #43116, .T. ) ;
#61460=AXIS2_PLACEMENT_3D ( 'NONE', #71763, #1716, #41034 ) ;
#61461=EDGE_CURVE ( 'NONE', #35080, #96401, #3583, .T. ) ;
#61463=EDGE_CURVE ( 'NONE', #105776, #58192, #18244, .T. ) ;
#61464=DIRECTION ( 'NONE',  ( -0.000000000000000000, 1.000000000000000000, -0.000000000000000000 ) ) ;
#61465=DIRECTION ( 'NONE',  ( -4.274815082592931898E-19, -0.9999939076577903929, -0.003490651415223739937 ) ) ;
#61466=EDGE_LOOP ( 'NONE', ( #52629, #122993, #31728, #102363 ) ) ;
#61467=DIRECTION ( 'NONE',  ( -0.000000000000000000, -1.000000000000000000, -0.000000000000000000 ) ) ;
#61468=CIRCLE ( 'NONE', #63514, 0.06509327318403741736 ) ;
#61469=CARTESIAN_POINT ( 'NONE',  ( -3.750000000000027534, 12.50000000000000000, -1.472243186433550122 ) ) ;
#61470=ORIENTED_EDGE ( 'NONE', *, *, #128910, .F. ) ;
#61471=AXIS2_PLACEMENT_3D ( 'NONE', #49909, #110098, #28974 ) ;
#61472=VECTOR ( 'NONE', #20540, 1000.000000000000000 ) ;
#61473=CIRCLE ( 'NONE', #904, 0.06509327318403745899 ) ;
#61474=VERTEX_POINT ( 'NONE', #73734 ) ;
#61475=EDGE_LOOP ( 'NONE', ( #110809, #82839, #34104, #34752 ) ) ;
#61476=ORIENTED_EDGE ( 'NONE', *, *, #76769, .T. ) ;
#61477=DIRECTION ( 'NONE',  ( 0.000000000000000000, 0.000000000000000000, -1.000000000000000000 ) ) ;
#61478=DIRECTION ( 'NONE',  ( 0.000000000000000000, 1.000000000000000000, 0.000000000000000000 ) ) ;
#61479=CARTESIAN_POINT ( 'NONE',  ( 2.500000000000001776, -2.021986658763283096, -9.892226903609810051 ) ) ;
#61480=AXIS2_PLACEMENT_3D ( 'NONE', #46191, #56634, #23986 ) ;
#61481=ORIENTED_EDGE ( 'NONE', *, *, #41363, .T. ) ;
#61482=DIRECTION ( 'NONE',  ( 0.000000000000000000, 1.000000000000000000, 0.000000000000000000 ) ) ;
#61483=ORIENTED_EDGE ( 'NONE', *, *, #128035, .T. ) ;
#61484=PLANE ( 'NONE',  #70526 ) ;
#61485=FACE_OUTER_BOUND ( 'NONE', #64610, .T. ) ;
#61486=LINE ( 'NONE', #92204, #111083 ) ;
#61487=CARTESIAN_POINT ( 'NONE',  ( -13.09999999999999254, 2.500000000000000000, -4.676537180435975216 ) ) ;
#61488=ORIENTED_EDGE ( 'NONE', *, *, #6494, .T. ) ;
#61489=ORIENTED_EDGE ( 'NONE', *, *, #68445, .F. ) ;
#61490=AXIS2_PLACEMENT_3D ( 'NONE', #92827, #3789, #101996 ) ;
#61491=ORIENTED_EDGE ( 'NONE', *, *, #20594, .T. ) ;
#61492=DIRECTION ( 'NONE',  ( -0.000000000000000000, -1.000000000000000000, -0.000000000000000000 ) ) ;
#61493=CONICAL_SURFACE ( 'NONE', #63635, 0.1000000000000002554, 0.003490658503988666988 ) ;
#61494=DIRECTION ( 'NONE',  ( -0.000000000000000000, 1.000000000000000000, -0.000000000000000000 ) ) ;
#61495=FACE_BOUND ( 'NONE', #10551, .T. ) ;
#61496=FACE_OUTER_BOUND ( 'NONE', #103282, .T. ) ;
#61497=CARTESIAN_POINT ( 'NONE',  ( 13.94999999999989804, 2.500000000000000000, 1.918653347947321564 ) ) ;
#61498=CARTESIAN_POINT ( 'NONE',  ( -2.499999999999996003, 2.500000000000000000, -4.230127018922201998 ) ) ;
#61499=EDGE_CURVE ( 'NONE', #120419, #120803, #122717, .T. ) ;
#61500=AXIS2_PLACEMENT_3D ( 'NONE', #76122, #47957, #56464 ) ;
#61501=AXIS2_PLACEMENT_3D ( 'NONE', #98591, #8289, #48226 ) ;
#61502=CONICAL_SURFACE ( 'NONE', #84471, 0.1000000000000002554, 0.003490658503988666988 ) ;
#61504=LINE ( 'NONE', #101415, #2411 ) ;
#61506=CARTESIAN_POINT ( 'NONE',  ( 11.24999999999994316, 2.500000000000000000, 2.265063509461097357 ) ) ;
#61507=ORIENTED_EDGE ( 'NONE', *, *, #29573, .F. ) ;
#61508=AXIS2_PLACEMENT_3D ( 'NONE', #69995, #2508, #41835 ) ;
#61509=CARTESIAN_POINT ( 'NONE',  ( 11.24999999999990941, 12.50000000000000000, 7.253104124594885960 ) ) ;
#61510=VECTOR ( 'NONE', #96961, 1000.000000000000000 ) ;
#61511=FACE_OUTER_BOUND ( 'NONE', #43459, .T. ) ;
#61513=EDGE_LOOP ( 'NONE', ( #113326, #4012 ) ) ;
#61514=CIRCLE ( 'NONE', #38537, 0.09999999999999999167 ) ;
#61515=EDGE_CURVE ( 'NONE', #8603, #79214, #21423, .T. ) ;
#61516=DIRECTION ( 'NONE',  ( 0.000000000000000000, 0.000000000000000000, -1.000000000000000000 ) ) ;
#61517=CARTESIAN_POINT ( 'NONE',  ( 6.849999999999930367, 2.500000000000000000, -6.148780366869526226 ) ) ;
#61518=EDGE_CURVE ( 'NONE', #26678, #38170, #99740, .T. ) ;
#61519=FACE_BOUND ( 'NONE', #34433, .T. ) ;
#61520=CARTESIAN_POINT ( 'NONE',  ( 15.83209681635555022, -2.500000000000000000, -5.404881881984138658 ) ) ;
#61522=ORIENTED_EDGE ( 'NONE', *, *, #77270, .F. ) ;
#61523=DIRECTION ( 'NONE',  ( 0.000000000000000000, 0.000000000000000000, -1.000000000000000000 ) ) ;
#61524=EDGE_CURVE ( 'NONE', #107, #5118, #64211, .T. ) ;
#61525=DIRECTION ( 'NONE',  ( 0.000000000000000000, 0.000000000000000000, 1.000000000000000000 ) ) ;
#61527=ORIENTED_EDGE ( 'NONE', *, *, #81185, .F. ) ;
#61528=CARTESIAN_POINT ( 'NONE',  ( -9.150000000000005684, 2.500000000000000000, 5.702370205355745014 ) ) ;
#61529=DIRECTION ( 'NONE',  ( -0.000000000000000000, -1.000000000000000000, -0.000000000000000000 ) ) ;
#61530=CARTESIAN_POINT ( 'NONE',  ( -2.500000000000032419, 2.500000000000000000, -3.737306695894649700 ) ) ;
#61531=CARTESIAN_POINT ( 'NONE',  ( -12.09999999999999609, 12.50000000000000000, 0.7579135962115910452 ) ) ;
#61532=CIRCLE ( 'NONE', #115802, 0.09999999999999982514 ) ;
#61533=EDGE_LOOP ( 'NONE', ( #61193, #55933, #83905, #84857 ) ) ;
#61534=CARTESIAN_POINT ( 'NONE',  ( -11.05000000000000249, 12.50000000000000000, -6.148780366869522673 ) ) ;
#61535=CARTESIAN_POINT ( 'NONE',  ( 8.749999999999953815, 2.500000000000000000, -2.165063509461101710 ) ) ;
#61536=DIRECTION ( 'NONE',  ( -0.000000000000000000, -1.000000000000000000, -0.000000000000000000 ) ) ;
#61537=ORIENTED_EDGE ( 'NONE', *, *, #67226, .T. ) ;
#61538=VERTEX_POINT ( 'NONE', #63285 ) ;
#61539=FACE_OUTER_BOUND ( 'NONE', #73632, .T. ) ;
#61540=EDGE_LOOP ( 'NONE', ( #37451, #8846 ) ) ;
#61541=DIRECTION ( 'NONE',  ( -4.274815082592931898E-19, -0.9999939076577903929, -0.003490651415223739937 ) ) ;
#61542=DIRECTION ( 'NONE',  ( 0.000000000000000000, 1.000000000000000000, 0.000000000000000000 ) ) ;
#61543=AXIS2_PLACEMENT_3D ( 'NONE', #47458, #67728, #38287 ) ;
#61544=EDGE_CURVE ( 'NONE', #26678, #50768, #112394, .T. ) ;
#61545=CARTESIAN_POINT ( 'NONE',  ( -10.40000000000000213, 2.500000000000000000, 0.5928203230275495006 ) ) ;
#61546=ORIENTED_EDGE ( 'NONE', *, *, #53248, .T. ) ;
#61547=CARTESIAN_POINT ( 'NONE',  ( -0.4000000000000331624, 2.500000000000000000, 0.000000000000000000 ) ) ;
#61548=DIRECTION ( 'NONE',  ( 0.000000000000000000, 1.000000000000000000, 0.000000000000000000 ) ) ;
#61549=CARTESIAN_POINT ( 'NONE',  ( 2.699999999999946443, 2.500000000000000000, 0.3464101615137735735 ) ) ;
#61550=CARTESIAN_POINT ( 'NONE',  ( -0.8500000000000386136, 12.50000000000000000, 2.922977105672686982 ) ) ;
#61551=DIRECTION ( 'NONE',  ( -4.274815082592931898E-19, -0.9999939076577903929, -0.003490651415223739937 ) ) ;
#61552=ADVANCED_FACE ( 'NONE', ( #103210 ), #108128, .T. ) ;
#61553=DIRECTION ( 'NONE',  ( -0.000000000000000000, -1.000000000000000000, -0.000000000000000000 ) ) ;
#61555=ORIENTED_EDGE ( 'NONE', *, *, #112938, .T. ) ;
#61556=ORIENTED_EDGE ( 'NONE', *, *, #23968, .T. ) ;
#61558=AXIS2_PLACEMENT_3D ( 'NONE', #80650, #1423, #123146 ) ;
#61559=ORIENTED_EDGE ( 'NONE', *, *, #69026, .F. ) ;
#61560=CIRCLE ( 'NONE', #17705, 0.1000000000000002554 ) ;
#61561=LINE ( 'NONE', #49813, #80697 ) ;
#61562=EDGE_CURVE ( 'NONE', #48575, #33637, #82939, .T. ) ;
#61563=ORIENTED_EDGE ( 'NONE', *, *, #87210, .F. ) ;
#61564=ORIENTED_EDGE ( 'NONE', *, *, #102339, .F. ) ;
#61565=EDGE_CURVE ( 'NONE', #2276, #12831, #87190, .T. ) ;
#61566=EDGE_LOOP ( 'NONE', ( #38636, #85931, #112592, #29932 ) ) ;
#61567=CIRCLE ( 'NONE', #11371, 0.1000000000000000056 ) ;
#61568=ADVANCED_FACE ( 'NONE', ( #33820 ), #82293, .T. ) ;
#61569=CARTESIAN_POINT ( 'NONE',  ( 5.799999999999934985, 2.500000000000000000, -4.330127018922201643 ) ) ;
#61570=EDGE_CURVE ( 'NONE', #112245, #115252, #76743, .T. ) ;
#61571=AXIS2_PLACEMENT_3D ( 'NONE', #9495, #39627, #107696 ) ;
#61572=FACE_OUTER_BOUND ( 'NONE', #62522, .T. ) ;
#61573=DIRECTION ( 'NONE',  ( 0.000000000000000000, 1.000000000000000000, 0.000000000000000000 ) ) ;
#61574=ADVANCED_FACE ( 'NONE', ( #62011 ), #20306, .T. ) ;
#61575=DIRECTION ( 'NONE',  ( -0.000000000000000000, -1.000000000000000000, -0.000000000000000000 ) ) ;
#61576=FACE_OUTER_BOUND ( 'NONE', #33096, .T. ) ;
#61577=CARTESIAN_POINT ( 'NONE',  ( 1.249999999999988454, 12.50000000000000000, 2.230156782645134950 ) ) ;
#61578=CARTESIAN_POINT ( 'NONE',  ( 1.249999999999953815, 2.500000000000000000, -2.757883832488654097 ) ) ;
#61579=DIRECTION ( 'NONE',  ( 0.000000000000000000, -0.9999939076577903929, 0.003490651415223739937 ) ) ;
#61580=DIRECTION ( 'NONE',  ( 0.000000000000000000, -0.000000000000000000, 1.000000000000000000 ) ) ;
#61581=EDGE_CURVE ( 'NONE', #23243, #87251, #62656, .T. ) ;
#61582=ORIENTED_EDGE ( 'NONE', *, *, #27261, .T. ) ;
#61583=CIRCLE ( 'NONE', #124262, 0.06509327318403745899 ) ;
#61584=CIRCLE ( 'NONE', #25976, 0.06509327318403745899 ) ;
#61585=DIRECTION ( 'NONE',  ( -0.000000000000000000, 1.000000000000000000, -0.000000000000000000 ) ) ;
#61586=AXIS2_PLACEMENT_3D ( 'NONE', #55452, #26002, #27270 ) ;
#61587=CIRCLE ( 'NONE', #107632, 0.1000000000000002554 ) ;
#61588=VERTEX_POINT ( 'NONE', #87425 ) ;
#61589=ORIENTED_EDGE ( 'NONE', *, *, #113232, .F. ) ;
#61590=CARTESIAN_POINT ( 'NONE',  ( -10.45000000000000107, 12.50000000000000000, 2.165063509461097713 ) ) ;
#61591=CARTESIAN_POINT ( 'NONE',  ( -2.100000000000034728, 2.500000000000000000, 4.230127018922196669 ) ) ;
#61592=CARTESIAN_POINT ( 'NONE',  ( -6.650000000000014566, 12.50000000000000000, 5.737276932171707422 ) ) ;
#61594=CONICAL_SURFACE ( 'NONE', #124277, 0.1000000000000002554, 0.003490658503988666988 ) ;
#61595=AXIS2_PLACEMENT_3D ( 'NONE', #104390, #64456, #94558 ) ;
#61596=DIRECTION ( 'NONE',  ( 0.000000000000000000, 1.000000000000000000, 0.000000000000000000 ) ) ;
#61597=DIRECTION ( 'NONE',  ( -0.000000000000000000, 1.000000000000000000, -0.000000000000000000 ) ) ;
#61598=DIRECTION ( 'NONE',  ( 0.000000000000000000, 1.000000000000000000, 0.000000000000000000 ) ) ;
#61599=ORIENTED_EDGE ( 'NONE', *, *, #103667, .F. ) ;
#61600=AXIS2_PLACEMENT_3D ( 'NONE', #88272, #107289, #49042 ) ;
#61601=ORIENTED_EDGE ( 'NONE', *, *, #84283, .T. ) ;
#61602=AXIS2_PLACEMENT_3D ( 'NONE', #11100, #23507, #80520 ) ;
#61603=EDGE_LOOP ( 'NONE', ( #107577, #66866, #48909, #99940 ) ) ;
#61604=ORIENTED_EDGE ( 'NONE', *, *, #37712, .F. ) ;
#61605=AXIS2_PLACEMENT_3D ( 'NONE', #77673, #116949, #47595 ) ;
#61606=EDGE_LOOP ( 'NONE', ( #93779, #129125, #44927, #93451 ) ) ;
#61607=CARTESIAN_POINT ( 'NONE',  ( 4.799999999999939426, 12.50000000000000000, -4.611443907251939756 ) ) ;
#61608=DIRECTION ( 'NONE',  ( -0.000000000000000000, -1.000000000000000000, -0.000000000000000000 ) ) ;
#61609=CARTESIAN_POINT ( 'NONE',  ( -12.09999999999999609, 2.500000000000000000, 4.430127018922196847 ) ) ;
#61610=EDGE_CURVE ( 'NONE', #4240, #103155, #67114, .T. ) ;
#61611=DIRECTION ( 'NONE',  ( -0.000000000000000000, -1.000000000000000000, -0.000000000000000000 ) ) ;
#61612=CARTESIAN_POINT ( 'NONE',  ( 9.599999999999917932, 2.500000000000000000, -2.276824562219559311E-15 ) ) ;
#61613=ORIENTED_EDGE ( 'NONE', *, *, #110465, .T. ) ;
#61614=CARTESIAN_POINT ( 'NONE',  ( 0.3999999999999619971, 12.50000000000000000, -1.084202172485504434E-16 ) ) ;
#61615=DIRECTION ( 'NONE',  ( 0.000000000000000000, 0.000000000000000000, -1.000000000000000000 ) ) ;
#61616=CARTESIAN_POINT ( 'NONE',  ( -10.85000000000000142, 12.50000000000000000, -6.495190528383298911 ) ) ;
#61617=CARTESIAN_POINT ( 'NONE',  ( -9.600000000000008527, 2.500000000000000000, -3.537306695894645969 ) ) ;
#61618=DIRECTION ( 'NONE',  ( 0.000000000000000000, 1.000000000000000000, 0.000000000000000000 ) ) ;
#61619=ADVANCED_FACE ( 'NONE', ( #116876 ), #28728, .T. ) ;
#61620=ORIENTED_EDGE ( 'NONE', *, *, #112026, .F. ) ;
#61621=VERTEX_POINT ( 'NONE', #74395 ) ;
#61622=VERTEX_POINT ( 'NONE', #105789 ) ;
#61623=CARTESIAN_POINT ( 'NONE',  ( -6.249999999999981348, 2.500000000000000000, 2.065063509461097624 ) ) ;
#61624=VERTEX_POINT ( 'NONE', #114318 ) ;
#61625=AXIS2_PLACEMENT_3D ( 'NONE', #5636, #126060, #64565 ) ;
#61626=CARTESIAN_POINT ( 'NONE',  ( 10.79999999999991367, 12.50000000000000000, 0.06509327318403504425 ) ) ;
#61628=CONICAL_SURFACE ( 'NONE', #5160, 0.1000000000000000472, 0.003490658503988666988 ) ;
#61629=ORIENTED_EDGE ( 'NONE', *, *, #59221, .T. ) ;
#61630=FACE_OUTER_BOUND ( 'NONE', #44893, .T. ) ;
#61631=DIRECTION ( 'NONE',  ( 0.000000000000000000, -0.9999939076577903929, 0.003490651415223739937 ) ) ;
#61632=DIRECTION ( 'NONE',  ( 0.000000000000000000, 1.000000000000000000, 0.000000000000000000 ) ) ;
#61633=CARTESIAN_POINT ( 'NONE',  ( -6.650000000000015454, 12.50000000000000000, 7.188010851410848723 ) ) ;
#61634=AXIS2_PLACEMENT_3D ( 'NONE', #89157, #101560, #128460 ) ;
#61635=DIRECTION ( 'NONE',  ( 0.000000000000000000, 0.000000000000000000, -1.000000000000000000 ) ) ;
#61636=CONICAL_SURFACE ( 'NONE', #70233, 0.09999999999999982514, 0.003490658503988666988 ) ;
#61637=ORIENTED_EDGE ( 'NONE', *, *, #27504, .T. ) ;
#61638=ORIENTED_EDGE ( 'NONE', *, *, #55778, .F. ) ;
#61639=DIRECTION ( 'NONE',  ( -4.274815082592931898E-19, -0.9999939076577903929, -0.003490651415223739937 ) ) ;
#61640=CARTESIAN_POINT ( 'NONE',  ( -9.999999999999969802, 12.50000000000000000, 0.06509327318403515528 ) ) ;
#61641=DIRECTION ( 'NONE',  ( 0.000000000000000000, 1.000000000000000000, 0.000000000000000000 ) ) ;
#61642=DIRECTION ( 'NONE',  ( -0.000000000000000000, 1.000000000000000000, -0.000000000000000000 ) ) ;
#61643=EDGE_CURVE ( 'NONE', #35451, #3120, #65195, .T. ) ;
#61644=ORIENTED_EDGE ( 'NONE', *, *, #96079, .F. ) ;
#61645=CONICAL_SURFACE ( 'NONE', #15642, 0.1000000000000002554, 0.003490658503988666988 ) ;
#61646=CONICAL_SURFACE ( 'NONE', #101359, 0.1000000000000002554, 0.003490658503988666988 ) ;
#61647=CIRCLE ( 'NONE', #74167, 0.1000000000000002554 ) ;
#61648=EDGE_LOOP ( 'NONE', ( #51929, #80594, #74744, #113253 ) ) ;
#61649=FACE_OUTER_BOUND ( 'NONE', #37428, .T. ) ;
#61650=FACE_OUTER_BOUND ( 'NONE', #129446, .T. ) ;
#61651=DIRECTION ( 'NONE',  ( 0.000000000000000000, -0.9999939076577903929, 0.003490651415223739937 ) ) ;
#61652=AXIS2_PLACEMENT_3D ( 'NONE', #59257, #37674, #99169 ) ;
#61653=DIRECTION ( 'NONE',  ( -4.274815082592931898E-19, -0.9999939076577903929, -0.003490651415223739937 ) ) ;
#61654=ORIENTED_EDGE ( 'NONE', *, *, #34196, .F. ) ;
#61655=EDGE_CURVE ( 'NONE', #45027, #180, #66271, .T. ) ;
#61656=DIRECTION ( 'NONE',  ( -0.000000000000000000, -1.000000000000000000, -0.000000000000000000 ) ) ;
#61657=DIRECTION ( 'NONE',  ( 0.000000000000000000, 1.000000000000000000, 0.000000000000000000 ) ) ;
#61658=EDGE_LOOP ( 'NONE', ( #72019, #62014, #125400, #111057 ) ) ;
#61659=EDGE_CURVE ( 'NONE', #90431, #76525, #101876, .T. ) ;
#61660=FACE_OUTER_BOUND ( 'NONE', #127779, .T. ) ;
#61661=ADVANCED_FACE ( 'NONE', ( #17384 ), #105133, .T. ) ;
#61662=EDGE_LOOP ( 'NONE', ( #24241, #41409 ) ) ;
#61663=CARTESIAN_POINT ( 'NONE',  ( 4.349999999999936584, 2.500000000000000000, 6.048780366869520364 ) ) ;
#61664=ORIENTED_EDGE ( 'NONE', *, *, #118697, .T. ) ;
#61665=CIRCLE ( 'NONE', #40748, 0.06509327318403745899 ) ;
#61666=ORIENTED_EDGE ( 'NONE', *, *, #87428, .T. ) ;
#61667=LINE ( 'NONE', #11903, #109181 ) ;
#61668=CARTESIAN_POINT ( 'NONE',  ( -14.59999999999998366, 2.500000000000000000, -0.6928203230275520319 ) ) ;
#61669=EDGE_CURVE ( 'NONE', #28566, #57456, #16733, .T. ) ;
#61670=CIRCLE ( 'NONE', #38603, 0.09999999999999982514 ) ;
#61671=AXIS2_PLACEMENT_3D ( 'NONE', #107737, #116256, #108377 ) ;
#61672=ORIENTED_EDGE ( 'NONE', *, *, #11201, .F. ) ;
#61673=ORIENTED_EDGE ( 'NONE', *, *, #116067, .T. ) ;
#61674=EDGE_CURVE ( 'NONE', #40266, #122166, #97253, .T. ) ;
#61675=CARTESIAN_POINT ( 'NONE',  ( 9.549999999999915445, 2.500000000000000000, 6.495190528383297135 ) ) ;
#61676=DIRECTION ( 'NONE',  ( 0.000000000000000000, 0.000000000000000000, 1.000000000000000000 ) ) ;
#61677=CARTESIAN_POINT ( 'NONE',  ( -2.300000000000032685, 2.500000000000000000, -0.4464101615137783252 ) ) ;
#61679=CONICAL_SURFACE ( 'NONE', #53269, 0.09999999999999982514, 0.003490658503988666988 ) ;
#61680=CIRCLE ( 'NONE', #124370, 0.06509327318403745899 ) ;
#61681=CARTESIAN_POINT ( 'NONE',  ( 14.54999999999989591, 12.50000000000000000, 2.165063509461097713 ) ) ;
#61682=LINE ( 'NONE', #51856, #126737 ) ;
#61683=FACE_OUTER_BOUND ( 'NONE', #23978, .T. ) ;
#61684=CONICAL_SURFACE ( 'NONE', #3191, 0.1000000000000002554, 0.003490658503988666988 ) ;
#61685=LINE ( 'NONE', #71477, #64037 ) ;
#61686=DIRECTION ( 'NONE',  ( 0.000000000000000000, 1.000000000000000000, 0.000000000000000000 ) ) ;
#61687=CIRCLE ( 'NONE', #53283, 0.06509327318403745899 ) ;
#61689=EDGE_LOOP ( 'NONE', ( #81297, #74842, #44199, #103682 ) ) ;
#61690=ORIENTED_EDGE ( 'NONE', *, *, #72061, .T. ) ;
#61691=PLANE ( 'NONE',  #69547 ) ;
#61692=EDGE_LOOP ( 'NONE', ( #117216, #94420 ) ) ;
#61693=CARTESIAN_POINT ( 'NONE',  ( -4.250072516143177381E-14, 2.500000000000000000, -3.637306695894650055 ) ) ;
#61694=CARTESIAN_POINT ( 'NONE',  ( 6.649999999999930189, 12.50000000000000000, -2.857883832488653741 ) ) ;
#61695=VECTOR ( 'NONE', #88463, 1000.000000000000000 ) ;
#61696=DIRECTION ( 'NONE',  ( 0.000000000000000000, 0.000000000000000000, -1.000000000000000000 ) ) ;
#61697=VERTEX_POINT ( 'NONE', #47522 ) ;
#61698=ORIENTED_EDGE ( 'NONE', *, *, #16732, .F. ) ;
#61699=FACE_BOUND ( 'NONE', #79898, .T. ) ;
#61700=ORIENTED_EDGE ( 'NONE', *, *, #30550, .F. ) ;
#61701=DIRECTION ( 'NONE',  ( -0.000000000000000000, 1.000000000000000000, -0.000000000000000000 ) ) ;
#61702=DIRECTION ( 'NONE',  ( 0.000000000000000000, 0.000000000000000000, 1.000000000000000000 ) ) ;
#61703=DIRECTION ( 'NONE',  ( 0.000000000000000000, 1.000000000000000000, 0.000000000000000000 ) ) ;
#61704=CARTESIAN_POINT ( 'NONE',  ( 2.299999999999947864, 2.500000000000000000, 4.083716857408421497 ) ) ;
#61705=LINE ( 'NONE', #101624, #70236 ) ;
#61706=DIRECTION ( 'NONE',  ( -0.000000000000000000, 1.000000000000000000, -0.000000000000000000 ) ) ;
#61707=DIRECTION ( 'NONE',  ( 0.000000000000000000, 1.000000000000000000, 0.000000000000000000 ) ) ;
#61708=DIRECTION ( 'NONE',  ( 0.000000000000000000, 1.000000000000000000, 0.000000000000000000 ) ) ;
#61709=FACE_OUTER_BOUND ( 'NONE', #54475, .T. ) ;
#61710=CARTESIAN_POINT ( 'NONE',  ( 10.64999999999991331, 12.50000000000000000, 6.841600689897072485 ) ) ;
#61711=AXIS2_PLACEMENT_3D ( 'NONE', #61694, #93084, #54422 ) ;
#61712=DIRECTION ( 'NONE',  ( 0.000000000000000000, 1.000000000000000000, 0.000000000000000000 ) ) ;
#61713=ADVANCED_FACE ( 'NONE', ( #127370 ), #55899, .T. ) ;
#61714=ORIENTED_EDGE ( 'NONE', *, *, #5126, .T. ) ;
#61715=ORIENTED_EDGE ( 'NONE', *, *, #93158, .T. ) ;
#61716=ORIENTED_EDGE ( 'NONE', *, *, #112615, .F. ) ;
#61717=ORIENTED_EDGE ( 'NONE', *, *, #93828, .F. ) ;
#61718=CARTESIAN_POINT ( 'NONE',  ( 11.44999999999990692, 12.50000000000000000, -6.841600689897078702 ) ) ;
#61719=EDGE_CURVE ( 'NONE', #1993, #54526, #5638, .T. ) ;
#61720=CARTESIAN_POINT ( 'NONE',  ( -9.600000000000008527, 2.500000000000000000, 4.330127018922196314 ) ) ;
#61721=EDGE_CURVE ( 'NONE', #13533, #40017, #118589, .T. ) ;
#61722=ORIENTED_EDGE ( 'NONE', *, *, #95399, .F. ) ;
#61723=ORIENTED_EDGE ( 'NONE', *, *, #50162, .T. ) ;
#61724=ORIENTED_EDGE ( 'NONE', *, *, #61659, .T. ) ;
#61725=EDGE_CURVE ( 'NONE', #118121, #89261, #49666, .T. ) ;
#61726=DIRECTION ( 'NONE',  ( 0.000000000000000000, 1.000000000000000000, 0.000000000000000000 ) ) ;
#61727=AXIS2_PLACEMENT_3D ( 'NONE', #30475, #129324, #79557 ) ;
#61728=ADVANCED_FACE ( 'NONE', ( #14794 ), #62178, .T. ) ;
#61729=VECTOR ( 'NONE', #29305, 1000.000000000000000 ) ;
#61730=CARTESIAN_POINT ( 'NONE',  ( 5.449999999999936229, 2.500000000000000000, -2.165063509461101710 ) ) ;
#61731=PRESENTATION_STYLE_ASSIGNMENT (( #91816 ) ) ;
#61732=CARTESIAN_POINT ( 'NONE',  ( -0.6000000000000323963, 12.50000000000000000, 0.2813168883297385570 ) ) ;
#61734=FACE_OUTER_BOUND ( 'NONE', #93496, .T. ) ;
#61735=DIRECTION ( 'NONE',  ( 0.000000000000000000, 1.000000000000000000, 0.000000000000000000 ) ) ;
#61736=DIRECTION ( 'NONE',  ( 0.000000000000000000, 0.000000000000000000, -1.000000000000000000 ) ) ;
#61738=DIRECTION ( 'NONE',  ( 0.000000000000000000, 1.000000000000000000, 0.000000000000000000 ) ) ;
#61739=EDGE_CURVE ( 'NONE', #62716, #42325, #72636, .T. ) ;
#61740=ORIENTED_EDGE ( 'NONE', *, *, #57300, .T. ) ;
#61741=CIRCLE ( 'NONE', #22025, 0.06509327318403745899 ) ;
#61742=ADVANCED_FACE ( 'NONE', ( #55403 ), #47503, .T. ) ;
#61743=ORIENTED_EDGE ( 'NONE', *, *, #67113, .T. ) ;
#61744=ORIENTED_EDGE ( 'NONE', *, *, #84002, .T. ) ;
#61745=CARTESIAN_POINT ( 'NONE',  ( -0.6000000000000383915, 2.500000000000000000, -4.083716857408426826 ) ) ;
#61746=ORIENTED_EDGE ( 'NONE', *, *, #57411, .T. ) ;
#61747=EDGE_LOOP ( 'NONE', ( #36371, #72227, #93420, #56777 ) ) ;
#61748=ORIENTED_EDGE ( 'NONE', *, *, #75548, .F. ) ;
#61749=CARTESIAN_POINT ( 'NONE',  ( -12.09999999999999609, 12.50000000000000000, -4.265033745738161741 ) ) ;
#61750=CONICAL_SURFACE ( 'NONE', #5276, 0.1000000000000002554, 0.003490658503988666988 ) ;
#61751=CARTESIAN_POINT ( 'NONE',  ( -9.150000000000005684, 12.50000000000000000, 7.122917578226811486 ) ) ;
#61752=AXIS2_PLACEMENT_3D ( 'NONE', #5478, #45433, #85346 ) ;
#61753=DIRECTION ( 'NONE',  ( -0.000000000000000000, -1.000000000000000000, -0.000000000000000000 ) ) ;
#61754=DIRECTION ( 'NONE',  ( 0.000000000000000000, 0.000000000000000000, -1.000000000000000000 ) ) ;
#61755=DIRECTION ( 'NONE',  ( 0.000000000000000000, 0.000000000000000000, -1.000000000000000000 ) ) ;
#61756=CARTESIAN_POINT ( 'NONE',  ( -14.59999999999998366, 12.50000000000000000, -0.6928203230275520319 ) ) ;
#61757=ORIENTED_EDGE ( 'NONE', *, *, #84108, .F. ) ;
#61758=CARTESIAN_POINT ( 'NONE',  ( 8.149999999999920419, 2.500000000000000000, -2.511473670974877948 ) ) ;
#61759=VERTEX_POINT ( 'NONE', #35762 ) ;
#61760=DIRECTION ( 'NONE',  ( -0.000000000000000000, 1.000000000000000000, -0.000000000000000000 ) ) ;
#61761=EDGE_LOOP ( 'NONE', ( #23742, #95682 ) ) ;
#61762=DIRECTION ( 'NONE',  ( -4.274815082592931898E-19, -0.9999939076577903929, -0.003490651415223739937 ) ) ;
#61763=CIRCLE ( 'NONE', #67995, 0.06509327318403745899 ) ;
#61764=ORIENTED_EDGE ( 'NONE', *, *, #125776, .T. ) ;
#61765=CARTESIAN_POINT ( 'NONE',  ( 14.14999999999989377, 2.500000000000000000, -2.757883832488654097 ) ) ;
#61766=CONICAL_SURFACE ( 'NONE', #72232, 0.1000000000000000472, 0.003490658503988666988 ) ;
#61767=AXIS2_PLACEMENT_3D ( 'NONE', #29717, #80113, #49382 ) ;
#61768=CARTESIAN_POINT ( 'NONE',  ( 4.549999999999939426, 2.500000000000000000, -2.265063509461101798 ) ) ;
#61769=ORIENTED_EDGE ( 'NONE', *, *, #22088, .T. ) ;
#61770=AXIS2_PLACEMENT_3D ( 'NONE', #81976, #53809, #22444 ) ;
#61771=ORIENTED_EDGE ( 'NONE', *, *, #6107, .F. ) ;
#61772=CARTESIAN_POINT ( 'NONE',  ( 9.549999999999918998, 2.500000000000000000, 2.065063509461097624 ) ) ;
#61773=CARTESIAN_POINT ( 'NONE',  ( -11.64999999999999680, 2.500000000000000000, 5.802370205355744659 ) ) ;
#61774=DIRECTION ( 'NONE',  ( -4.274815082592931898E-19, -0.9999939076577903929, -0.003490651415223739937 ) ) ;
#61775=CARTESIAN_POINT ( 'NONE',  ( -0.6000000000000323963, 12.50000000000000000, -0.2813168883297385570 ) ) ;
#61776=AXIS2_PLACEMENT_3D ( 'NONE', #26967, #128412, #38746 ) ;
#61777=DIRECTION ( 'NONE',  ( -0.000000000000000000, -1.000000000000000000, -0.000000000000000000 ) ) ;
#61778=ADVANCED_FACE ( 'NONE', ( #115590 ), #25947, .T. ) ;
#61779=CONICAL_SURFACE ( 'NONE', #111937, 0.1000000000000002554, 0.003490658503988666988 ) ;
#61780=EDGE_LOOP ( 'NONE', ( #29546, #67352 ) ) ;
#61781=CIRCLE ( 'NONE', #17835, 0.06509327318403745899 ) ;
#61782=CARTESIAN_POINT ( 'NONE',  ( -5.850000000000018296, 2.500000000000000000, 5.702370205355745014 ) ) ;
#61783=ORIENTED_EDGE ( 'NONE', *, *, #77752, .T. ) ;
#61785=DIRECTION ( 'NONE',  ( 0.000000000000000000, -0.9999939076577903929, 0.003490651415223739937 ) ) ;
#61786=VECTOR ( 'NONE', #64254, 1000.000000000000000 ) ;
#61787=AXIS2_PLACEMENT_3D ( 'NONE', #89875, #80720, #195 ) ;
#61788=VECTOR ( 'NONE', #125651, 1000.000000000000000 ) ;
#61790=CARTESIAN_POINT ( 'NONE',  ( 0.4499999999999552136, 2.500000000000000000, 6.595190528383296780 ) ) ;
#61791=LINE ( 'NONE', #83358, #73746 ) ;
#61793=DIRECTION ( 'NONE',  ( 0.000000000000000000, 0.000000000000000000, 1.000000000000000000 ) ) ;
#61794=ORIENTED_EDGE ( 'NONE', *, *, #476, .T. ) ;
#61795=FACE_OUTER_BOUND ( 'NONE', #100207, .T. ) ;
#61796=DIRECTION ( 'NONE',  ( 0.000000000000000000, 1.000000000000000000, 0.000000000000000000 ) ) ;
#61797=CARTESIAN_POINT ( 'NONE',  ( -13.54999999999999005, 2.500000000000000000, -1.818653347947323917 ) ) ;
#61798=ORIENTED_EDGE ( 'NONE', *, *, #93164, .T. ) ;
#61799=VECTOR ( 'NONE', #86457, 1000.000000000000000 ) ;
#61800=ORIENTED_EDGE ( 'NONE', *, *, #124663, .F. ) ;
#61801=CARTESIAN_POINT ( 'NONE',  ( -3.150000000000030553, 2.500000000000000000, 6.148780366869520009 ) ) ;
#61802=ORIENTED_EDGE ( 'NONE', *, *, #121067, .T. ) ;
#61803=EDGE_LOOP ( 'NONE', ( #24716, #76737 ) ) ;
#61804=FACE_OUTER_BOUND ( 'NONE', #78049, .T. ) ;
#61805=ORIENTED_EDGE ( 'NONE', *, *, #33169, .T. ) ;
#61806=CARTESIAN_POINT ( 'NONE',  ( 16.84158739989841180, -0.4722467112506605336, -5.802037699235492063 ) ) ;
#61807=EDGE_CURVE ( 'NONE', #122474, #112402, #103935, .T. ) ;
#61808=DIRECTION ( 'NONE',  ( -0.000000000000000000, -1.000000000000000000, -0.000000000000000000 ) ) ;
#61809=CARTESIAN_POINT ( 'NONE',  ( 17.17539648375905870, 2.541523116374017732, 5.507477068182278224 ) ) ;
#61810=AXIS2_PLACEMENT_3D ( 'NONE', #9370, #107573, #57834 ) ;
#61811=CONICAL_SURFACE ( 'NONE', #5353, 0.1000000000000002554, 0.003490658503988666988 ) ;
#61812=ORIENTED_EDGE ( 'NONE', *, *, #14651, .F. ) ;
#61813=ADVANCED_FACE ( 'NONE', ( #119460 ), #60134, .T. ) ;
#61815=CARTESIAN_POINT ( 'NONE',  ( 6.899999999999926636, 12.50000000000000000, -0.3464101615137782364 ) ) ;
#61816=ADVANCED_FACE ( 'NONE', ( #100478 ), #66449, .T. ) ;
#61817=EDGE_CURVE ( 'NONE', #16509, #120005, #30885, .T. ) ;
#61818=ORIENTED_EDGE ( 'NONE', *, *, #5818, .T. ) ;
#61819=CIRCLE ( 'NONE', #36785, 0.09999999999999982514 ) ;
#61820=ORIENTED_EDGE ( 'NONE', *, *, #98170, .F. ) ;
#61822=ORIENTED_EDGE ( 'NONE', *, *, #29572, .T. ) ;
#61823=CARTESIAN_POINT ( 'NONE',  ( 1.449999999999949551, 12.50000000000000000, 6.841600689897072485 ) ) ;
#61825=EDGE_CURVE ( 'NONE', #49326, #116833, #104023, .T. ) ;
#61826=ADVANCED_FACE ( 'NONE', ( #60582 ), #47598, .T. ) ;
#61827=DIRECTION ( 'NONE',  ( 0.000000000000000000, 0.000000000000000000, -1.000000000000000000 ) ) ;
#61828=ADVANCED_FACE ( 'NONE', ( #98522 ), #7862, .T. ) ;
#61829=FACE_BOUND ( 'NONE', #15169, .T. ) ;
#61830=ORIENTED_EDGE ( 'NONE', *, *, #87493, .F. ) ;
#61831=EDGE_CURVE ( 'NONE', #92562, #48804, #55980, .T. ) ;
#61832=CARTESIAN_POINT ( 'NONE',  ( 11.84999999999990727, 12.50000000000000000, -2.511473670974877948 ) ) ;
#61833=DIRECTION ( 'NONE',  ( 0.000000000000000000, 0.000000000000000000, -1.000000000000000000 ) ) ;
#61834=ORIENTED_EDGE ( 'NONE', *, *, #9216, .T. ) ;
#61835=CARTESIAN_POINT ( 'NONE',  ( 8.749999999999921840, 12.50000000000000000, 2.857883832488649301 ) ) ;
#61836=CARTESIAN_POINT ( 'NONE',  ( 0.8499999999999553468, 12.50000000000000000, -2.165063509461101710 ) ) ;
#61838=DIRECTION ( 'NONE',  ( -0.000000000000000000, 1.000000000000000000, -0.000000000000000000 ) ) ;
#61839=DIRECTION ( 'NONE',  ( -0.000000000000000000, 1.000000000000000000, -0.000000000000000000 ) ) ;
#61840=EDGE_CURVE ( 'NONE', #105625, #116790, #99830, .T. ) ;
#61841=LINE ( 'NONE', #40925, #32578 ) ;
#61842=DIRECTION ( 'NONE',  ( 0.000000000000000000, 1.000000000000000000, 0.000000000000000000 ) ) ;
#61843=EDGE_LOOP ( 'NONE', ( #79897, #97985, #42614, #91007 ) ) ;
#61844=ORIENTED_EDGE ( 'NONE', *, *, #13656, .F. ) ;
#61845=EDGE_LOOP ( 'NONE', ( #129141, #25413, #64876, #100826 ) ) ;
#61846=ORIENTED_EDGE ( 'NONE', *, *, #67618, .F. ) ;
#61847=CARTESIAN_POINT ( 'NONE',  ( 14.99999999999992895, 12.50000000000000000, -2.276824562219559311E-15 ) ) ;
#61848=DIRECTION ( 'NONE',  ( 0.000000000000000000, 0.000000000000000000, -1.000000000000000000 ) ) ;
#61849=ORIENTED_EDGE ( 'NONE', *, *, #93266, .T. ) ;
#61850=FACE_BOUND ( 'NONE', #33592, .T. ) ;
#61851=CARTESIAN_POINT ( 'NONE',  ( 11.04999999999990834, 2.500000000000000000, -6.841600689897077814 ) ) ;
#61852=CARTESIAN_POINT ( 'NONE',  ( -6.700000000000019718, 2.500000000000000000, -2.385244779468109755E-15 ) ) ;
#61853=CARTESIAN_POINT ( 'NONE',  ( -6.850000000000013856, 2.500000000000000000, 6.048780366869521252 ) ) ;
#61854=LINE ( 'NONE', #113512, #93034 ) ;
#61855=AXIS2_PLACEMENT_3D ( 'NONE', #118091, #109574, #79480 ) ;
#61856=DIRECTION ( 'NONE',  ( 0.000000000000000000, 1.000000000000000000, 0.000000000000000000 ) ) ;
#61857=CARTESIAN_POINT ( 'NONE',  ( 12.69999999999990159, 2.500000000000000000, -3.983716857408426293 ) ) ;
#61858=CARTESIAN_POINT ( 'NONE',  ( 3.349999999999945466, 2.500000000000000000, -2.165063509461101710 ) ) ;
#61859=CARTESIAN_POINT ( 'NONE',  ( 4.799999999999937650, 2.500000000000000000, -3.983716857408426293 ) ) ;
#61860=ADVANCED_FACE ( 'NONE', ( #27872 ), #118184, .T. ) ;
#61861=DIRECTION ( 'NONE',  ( -0.000000000000000000, -1.000000000000000000, -0.000000000000000000 ) ) ;
#61862=ORIENTED_EDGE ( 'NONE', *, *, #72895, .F. ) ;
#61863=ORIENTED_EDGE ( 'NONE', *, *, #28440, .F. ) ;
#61864=VERTEX_POINT ( 'NONE', #108362 ) ;
#61865=EDGE_LOOP ( 'NONE', ( #4703, #96253, #76397, #48152 ) ) ;
#61867=VERTEX_POINT ( 'NONE', #323 ) ;
#61868=VERTEX_POINT ( 'NONE', #129325 ) ;
#61869=CONICAL_SURFACE ( 'NONE', #28413, 0.09999999999999982514, 0.003490658503988666988 ) ;
#61870=CARTESIAN_POINT ( 'NONE',  ( -11.84999999999999787, 2.500000000000000000, -1.818653347947321919 ) ) ;
#61871=EDGE_CURVE ( 'NONE', #121723, #90081, #93555, .T. ) ;
#61872=VERTEX_POINT ( 'NONE', #69732 ) ;
#61874=EDGE_CURVE ( 'NONE', #27091, #70439, #120744, .T. ) ;
#61875=AXIS2_PLACEMENT_3D ( 'NONE', #27143, #67037, #17286 ) ;
#61876=VECTOR ( 'NONE', #106750, 1000.000000000000000 ) ;
#61877=ADVANCED_FACE ( 'NONE', ( #88726 ), #37135, .T. ) ;
#61878=AXIS2_PLACEMENT_3D ( 'NONE', #45949, #85844, #125760 ) ;
#61879=CARTESIAN_POINT ( 'NONE',  ( -6.249999999999984901, 2.500000000000000000, -2.065063509461102065 ) ) ;
#61880=CARTESIAN_POINT ( 'NONE',  ( 15.22989033368280154, -2.499999999999999556, 7.180069491320001163 ) ) ;
#61881=CARTESIAN_POINT ( 'NONE',  ( 8.549999999999924327, 12.50000000000000000, 1.818653347947321475 ) ) ;
#61882=CARTESIAN_POINT ( 'NONE',  ( 0.3999999999999568345, 2.500000000000000000, -5.022947341949754119 ) ) ;
#61883=AXIS2_PLACEMENT_3D ( 'NONE', #5086, #3810, #83667 ) ;
#61884=EDGE_CURVE ( 'NONE', #7480, #112355, #51803, .T. ) ;
#61885=ORIENTED_EDGE ( 'NONE', *, *, #84591, .F. ) ;
#61886=CARTESIAN_POINT ( 'NONE',  ( 8.949999999999915801, 2.500000000000000000, -1.718653347947326049 ) ) ;
#61887=EDGE_CURVE ( 'NONE', #72458, #37153, #79001, .T. ) ;
#61888=EDGE_CURVE ( 'NONE', #35194, #60040, #50113, .T. ) ;
#61889=ORIENTED_EDGE ( 'NONE', *, *, #106635, .T. ) ;
#61890=EDGE_CURVE ( 'NONE', #127833, #65132, #110280, .T. ) ;
#61891=ORIENTED_EDGE ( 'NONE', *, *, #57991, .F. ) ;
#61892=FACE_OUTER_BOUND ( 'NONE', #3805, .T. ) ;
#61893=DIRECTION ( 'NONE',  ( 0.000000000000000000, 0.000000000000000000, 1.000000000000000000 ) ) ;
#61894=AXIS2_PLACEMENT_3D ( 'NONE', #21598, #73919, #11770 ) ;
#61895=VERTEX_POINT ( 'NONE', #32420 ) ;
#61896=EDGE_CURVE ( 'NONE', #90044, #80196, #64308, .T. ) ;
#61897=ORIENTED_EDGE ( 'NONE', *, *, #54109, .F. ) ;
#61899=DIRECTION ( 'NONE',  ( 0.000000000000000000, 0.000000000000000000, -1.000000000000000000 ) ) ;
#61900=DIRECTION ( 'NONE',  ( 0.000000000000000000, 0.000000000000000000, 1.000000000000000000 ) ) ;
#61901=DIRECTION ( 'NONE',  ( 0.000000000000000000, 1.000000000000000000, 0.000000000000000000 ) ) ;
#61902=CARTESIAN_POINT ( 'NONE',  ( -3.100000000000028511, 12.50000000000000000, -0.4115034346978156399 ) ) ;
#61903=AXIS2_PLACEMENT_3D ( 'NONE', #28855, #86465, #126402 ) ;
#61904=AXIS2_PLACEMENT_3D ( 'NONE', #27675, #67604, #44771 ) ;
#61905=ORIENTED_EDGE ( 'NONE', *, *, #95679, .F. ) ;
#61906=CARTESIAN_POINT ( 'NONE',  ( 3.349999999999944578, 2.500000000000000000, -5.902370205355750521 ) ) ;
#61907=AXIS2_PLACEMENT_3D ( 'NONE', #115396, #125879, #15272 ) ;
#61908=ORIENTED_EDGE ( 'NONE', *, *, #44710, .F. ) ;
#61909=AXIS2_PLACEMENT_3D ( 'NONE', #108658, #1284, #79219 ) ;
#61910=DIRECTION ( 'NONE',  ( 0.000000000000000000, 0.000000000000000000, 1.000000000000000000 ) ) ;
#61911=FACE_OUTER_BOUND ( 'NONE', #75267, .T. ) ;
#61912=CARTESIAN_POINT ( 'NONE',  ( 4.799999999999939426, 12.50000000000000000, -4.676537180435977881 ) ) ;
#61913=CARTESIAN_POINT ( 'NONE',  ( 2.699999999999947331, 2.500000000000000000, -0.2464101615137783419 ) ) ;
#61914=DIRECTION ( 'NONE',  ( 0.000000000000000000, 0.000000000000000000, 1.000000000000000000 ) ) ;
#61915=ORIENTED_EDGE ( 'NONE', *, *, #24759, .F. ) ;
#61916=AXIS2_PLACEMENT_3D ( 'NONE', #89497, #49590, #100590 ) ;
#61917=LINE ( 'NONE', #112934, #94888 ) ;
#61918=VECTOR ( 'NONE', #41280, 1000.000000000000000 ) ;
#61920=PLANE ( 'NONE',  #52794 ) ;
#61921=ORIENTED_EDGE ( 'NONE', *, *, #96216, .F. ) ;
#61922=EDGE_LOOP ( 'NONE', ( #63887, #106039 ) ) ;
#61923=EDGE_LOOP ( 'NONE', ( #53291, #47426 ) ) ;
#61924=CARTESIAN_POINT ( 'NONE',  ( 14.99999999999989164, 2.500000000000000000, 0.6928203230275494784 ) ) ;
#61925=DIRECTION ( 'NONE',  ( -0.000000000000000000, 1.000000000000000000, -0.000000000000000000 ) ) ;
#61926=DIRECTION ( 'NONE',  ( 0.000000000000000000, 0.000000000000000000, 1.000000000000000000 ) ) ;
#61927=DIRECTION ( 'NONE',  ( 0.000000000000000000, -0.9999939076577903929, 0.003490651415223739937 ) ) ;
#61928=DIRECTION ( 'NONE',  ( 0.000000000000000000, 0.000000000000000000, -1.000000000000000000 ) ) ;
#61929=FACE_OUTER_BOUND ( 'NONE', #21582, .T. ) ;
#61930=ADVANCED_FACE ( 'NONE', ( #52666 ), #42217, .T. ) ;
#61931=CARTESIAN_POINT ( 'NONE',  ( -12.69999999999999218, 2.500000000000000000, 4.776537180435972196 ) ) ;
#61932=DIRECTION ( 'NONE',  ( -0.000000000000000000, 1.000000000000000000, -0.000000000000000000 ) ) ;
#61933=EDGE_LOOP ( 'NONE', ( #107813, #52389, #114838, #114584 ) ) ;
#61935=EDGE_CURVE ( 'NONE', #123233, #50100, #72723, .T. ) ;
#61936=CARTESIAN_POINT ( 'NONE',  ( -9.200000000000006395, 2.500000000000000000, -2.385244779468109755E-15 ) ) ;
#61937=DIRECTION ( 'NONE',  ( 0.000000000000000000, 0.000000000000000000, -1.000000000000000000 ) ) ;
#61938=DIRECTION ( 'NONE',  ( 0.000000000000000000, 1.000000000000000000, 0.000000000000000000 ) ) ;
#61939=ORIENTED_EDGE ( 'NONE', *, *, #17211, .T. ) ;
#61940=CARTESIAN_POINT ( 'NONE',  ( -8.749999999999975131, 2.500000000000000000, -2.165063509461101710 ) ) ;
#61941=CIRCLE ( 'NONE', #13791, 0.1000000000000002554 ) ;
#61942=CIRCLE ( 'NONE', #68179, 0.06509327318403745899 ) ;
#61943=DIRECTION ( 'NONE',  ( 0.000000000000000000, 0.000000000000000000, -1.000000000000000000 ) ) ;
#61944=DIRECTION ( 'NONE',  ( 0.000000000000000000, 0.000000000000000000, -1.000000000000000000 ) ) ;
#61945=ORIENTED_EDGE ( 'NONE', *, *, #27989, .F. ) ;
#61946=VERTEX_POINT ( 'NONE', #53331 ) ;
#61947=AXIS2_PLACEMENT_3D ( 'NONE', #69652, #42135, #91233 ) ;
#61948=AXIS2_PLACEMENT_3D ( 'NONE', #119601, #1755, #1121 ) ;
#61950=ORIENTED_EDGE ( 'NONE', *, *, #46424, .F. ) ;
#61951=ORIENTED_EDGE ( 'NONE', *, *, #67031, .F. ) ;
#61952=DIRECTION ( 'NONE',  ( 0.000000000000000000, 1.000000000000000000, 0.000000000000000000 ) ) ;
#61954=FACE_OUTER_BOUND ( 'NONE', #67363, .T. ) ;
#61955=CIRCLE ( 'NONE', #93261, 0.1000000000000000472 ) ;
#61956=CIRCLE ( 'NONE', #5499, 0.06509327318403745899 ) ;
#61957=CARTESIAN_POINT ( 'NONE',  ( 5.649999999999934630, 2.500000000000000000, -1.718653347947325827 ) ) ;
#61958=ORIENTED_EDGE ( 'NONE', *, *, #12608, .F. ) ;
#61959=CIRCLE ( 'NONE', #15963, 0.09999999999999982514 ) ;
#61960=EDGE_CURVE ( 'NONE', #91248, #80232, #113520, .T. ) ;
#61961=DIRECTION ( 'NONE',  ( 0.000000000000000000, 1.000000000000000000, 0.000000000000000000 ) ) ;
#61962=VERTEX_POINT ( 'NONE', #91303 ) ;
#61963=CARTESIAN_POINT ( 'NONE',  ( 8.299999999999922551, 2.500000000000000000, 4.330127018922196314 ) ) ;
#61964=EDGE_CURVE ( 'NONE', #113935, #27857, #22568, .T. ) ;
#61965=ORIENTED_EDGE ( 'NONE', *, *, #70021, .T. ) ;
#61966=ORIENTED_EDGE ( 'NONE', *, *, #13698, .T. ) ;
#61967=ORIENTED_EDGE ( 'NONE', *, *, #78244, .T. ) ;
#61968=ORIENTED_EDGE ( 'NONE', *, *, #35840, .T. ) ;
#61969=CARTESIAN_POINT ( 'NONE',  ( 0.3999999999999619971, 2.500000000000000000, 0.09999999999999989453 ) ) ;
#61970=CARTESIAN_POINT ( 'NONE',  ( 14.69113575703644869, 2.500000000000000000, 6.337000354879313235 ) ) ;
#61971=EDGE_CURVE ( 'NONE', #90560, #4778, #81050, .T. ) ;
#61972=ADVANCED_FACE ( 'NONE', ( #110929 ), #12095, .T. ) ;
#61973=CARTESIAN_POINT ( 'NONE',  ( -1.900000000000034106, 12.50000000000000000, 0.2813168883297361700 ) ) ;
#61974=ADVANCED_FACE ( 'NONE', ( #23868 ), #12074, .T. ) ;
#61975=FACE_BOUND ( 'NONE', #81377, .T. ) ;
#61976=VERTEX_POINT ( 'NONE', #1626 ) ;
#61977=EDGE_CURVE ( 'NONE', #94015, #18162, #31120, .T. ) ;
#61978=DIRECTION ( 'NONE',  ( 0.000000000000000000, 0.000000000000000000, -1.000000000000000000 ) ) ;
#61979=AXIS2_PLACEMENT_3D ( 'NONE', #89537, #77766, #99372 ) ;
#61981=DIRECTION ( 'NONE',  ( -0.000000000000000000, 1.000000000000000000, -0.000000000000000000 ) ) ;
#61982=DIRECTION ( 'NONE',  ( -0.000000000000000000, -1.000000000000000000, -0.000000000000000000 ) ) ;
#61983=AXIS2_PLACEMENT_3D ( 'NONE', #25229, #105080, #15409 ) ;
#61984=AXIS2_PLACEMENT_3D ( 'NONE', #6805, #5537, #76874 ) ;
#61985=DIRECTION ( 'NONE',  ( 0.000000000000000000, 1.000000000000000000, 0.000000000000000000 ) ) ;
#61986=PLANE ( 'NONE',  #25940 ) ;
#61988=CARTESIAN_POINT ( 'NONE',  ( -9.150000000000011013, 2.500000000000000000, -5.702370205355745014 ) ) ;
#61989=AXIS2_PLACEMENT_3D ( 'NONE', #85166, #125093, #35438 ) ;
#61990=AXIS2_PLACEMENT_3D ( 'NONE', #80674, #110755, #1449 ) ;
#61991=ADVANCED_FACE ( 'NONE', ( #43517 ), #122903, .T. ) ;
#61992=ADVANCED_FACE ( 'NONE', ( #72328 ), #45541, .T. ) ;
#61993=CARTESIAN_POINT ( 'NONE',  ( 12.09999999999990550, 2.500000000000000000, -3.737306695894649700 ) ) ;
#61994=CONICAL_SURFACE ( 'NONE', #7594, 0.1000000000000002554, 0.003490658503988666988 ) ;
#61995=EDGE_LOOP ( 'NONE', ( #2901, #69380, #9464, #18119 ) ) ;
#61996=ORIENTED_EDGE ( 'NONE', *, *, #121073, .T. ) ;
#61998=ORIENTED_EDGE ( 'NONE', *, *, #42610, .T. ) ;
#61999=ORIENTED_EDGE ( 'NONE', *, *, #38811, .F. ) ;
#62000=CARTESIAN_POINT ( 'NONE',  ( 11.69999999999990870, 2.500000000000000000, 4.330127018922196314 ) ) ;
#62001=CARTESIAN_POINT ( 'NONE',  ( 0.3999999999999563904, 12.50000000000000000, 3.637306695894644726 ) ) ;
#62002=VERTEX_POINT ( 'NONE', #33679 ) ;
#62003=FACE_BOUND ( 'NONE', #3438, .T. ) ;
#62004=CIRCLE ( 'NONE', #116356, 0.1000000000000002554 ) ;
#62005=DIRECTION ( 'NONE',  ( 0.000000000000000000, 1.000000000000000000, 0.000000000000000000 ) ) ;
#62006=AXIS2_PLACEMENT_3D ( 'NONE', #10356, #90850, #68625 ) ;
#62007=VECTOR ( 'NONE', #94357, 1000.000000000000000 ) ;
#62009=CARTESIAN_POINT ( 'NONE',  ( 2.899999999999943956, 2.500000000000000000, 4.430127018922196847 ) ) ;
#62010=CARTESIAN_POINT ( 'NONE',  ( -11.64999999999999680, 12.50000000000000000, 6.495190528383297135 ) ) ;
#62011=FACE_OUTER_BOUND ( 'NONE', #117984, .T. ) ;
#62012=ORIENTED_EDGE ( 'NONE', *, *, #86678, .T. ) ;
#62013=DIRECTION ( 'NONE',  ( -4.274815082592931898E-19, -0.9999939076577903929, -0.003490651415223739937 ) ) ;
#62014=ORIENTED_EDGE ( 'NONE', *, *, #118887, .F. ) ;
#62015=ORIENTED_EDGE ( 'NONE', *, *, #41790, .F. ) ;
#62016=VERTEX_POINT ( 'NONE', #83434 ) ;
#62017=DIRECTION ( 'NONE',  ( 0.000000000000000000, -0.000000000000000000, 1.000000000000000000 ) ) ;
#62018=DIRECTION ( 'NONE',  ( 0.000000000000000000, 0.000000000000000000, 1.000000000000000000 ) ) ;
#62019=EDGE_LOOP ( 'NONE', ( #69891, #71035, #116243, #67884 ) ) ;
#62020=LINE ( 'NONE', #12250, #80962 ) ;
#62022=CARTESIAN_POINT ( 'NONE',  ( 7.099999999999925926, 12.50000000000000000, 0.6928203230275494784 ) ) ;
#62023=DIRECTION ( 'NONE',  ( 0.000000000000000000, 1.000000000000000000, 0.000000000000000000 ) ) ;
#62025=ORIENTED_EDGE ( 'NONE', *, *, #22255, .F. ) ;
#62026=DIRECTION ( 'NONE',  ( -0.000000000000000000, -1.000000000000000000, -0.000000000000000000 ) ) ;
#62027=EDGE_CURVE ( 'NONE', #106414, #34384, #58065, .T. ) ;
#62028=ORIENTED_EDGE ( 'NONE', *, *, #116669, .F. ) ;
#62029=CARTESIAN_POINT ( 'NONE',  ( 10.39999999999991154, 2.500000000000000000, -3.537306695894649966 ) ) ;
#62030=EDGE_CURVE ( 'NONE', #46732, #24133, #40946, .T. ) ;
#62031=AXIS2_PLACEMENT_3D ( 'NONE', #123044, #102736, #104044 ) ;
#62032=ORIENTED_EDGE ( 'NONE', *, *, #108036, .F. ) ;
#62033=AXIS2_PLACEMENT_3D ( 'NONE', #42470, #100712, #112489 ) ;
#62034=CARTESIAN_POINT ( 'NONE',  ( -5.850000000000018296, 12.50000000000000000, 5.802370205355744659 ) ) ;
#62035=EDGE_CURVE ( 'NONE', #30567, #28910, #71029, .T. ) ;
#62036=VERTEX_POINT ( 'NONE', #81493 ) ;
#62039=( BOUNDED_SURFACE ( )  B_SPLINE_SURFACE ( 3, 2, ( 
 ( #81442, #23151, #108467 ),
 ( #8972, #12673, #63080 ),
 ( #62453, #52609, #112831 ),
 ( #102370, #71606, #120713 ),
 ( #111537, #18796, #2878 ),
 ( #128790, #2210, #93197 ),
 ( #91253, #58737, #39123 ),
 ( #78389, #98636, #51353 ),
 ( #32369, #1572, #31693 ),
 ( #102994, #13321, #80802 ),
 ( #53277, #92532, #3518 ),
 ( #118294, #121348, #61806 ),
 ( #48927, #82071, #28638 ),
 ( #61149, #72273, #72905 ) ),
 .UNSPECIFIED., .F., .F., .T. ) 
 B_SPLINE_SURFACE_WITH_KNOTS ( ( 4, 2, 2, 2, 2, 2, 4 ),
 ( 3, 3 ),
 ( 0.000000000000000000, 0.001744612550437227034, 0.002616918825655840768, 0.003489225100874454068, 0.005233837651311681535, 0.006106143926530294835, 0.006978450201748908135 ),
 ( 0.000000000000000000, 1.000000000000000000 ),
 .UNSPECIFIED. ) 
 GEOMETRIC_REPRESENTATION_ITEM ( )  RATIONAL_B_SPLINE_SURFACE ( (
 ( 1.000000000000000000, 0.7318752858502194369, 1.000000000000000000),
 ( 1.000000000000000000, 0.7270130115583837149, 1.000000000000000000),
 ( 1.000000000000000000, 0.7223762446132400150, 1.000000000000000000),
 ( 1.000000000000000000, 0.7156127915554295615, 1.000000000000000000),
 ( 1.000000000000000000, 0.7133893117690700558, 1.000000000000000000),
 ( 1.000000000000000000, 0.7090389252574490486, 1.000000000000000000),
 ( 1.000000000000000000, 0.7069297463491782674, 1.000000000000000000),
 ( 1.000000000000000000, 0.7010696893198986590, 1.000000000000000000),
 ( 1.000000000000000000, 0.6977361265597721296, 1.000000000000000000),
 ( 1.000000000000000000, 0.6948030504688549325, 1.000000000000000000),
 ( 1.000000000000000000, 0.6942033558615769984, 1.000000000000000000),
 ( 1.000000000000000000, 0.6937817651808135810, 1.000000000000000000),
 ( 1.000000000000000000, 0.6939284133497518603, 1.000000000000000000),
 ( 1.000000000000000000, 0.6944177883068419765, 1.000000000000000000) ) ) 
 REPRESENTATION_ITEM ( '' )  SURFACE ( )  );
#62040=FACE_OUTER_BOUND ( 'NONE', #14380, .T. ) ;
#62041=FACE_OUTER_BOUND ( 'NONE', #108349, .T. ) ;
#62042=FACE_OUTER_BOUND ( 'NONE', #10284, .T. ) ;
#62043=EDGE_LOOP ( 'NONE', ( #111356, #65420 ) ) ;
#62044=EDGE_CURVE ( 'NONE', #15792, #100531, #91500, .T. ) ;
#62045=AXIS2_PLACEMENT_3D ( 'NONE', #44556, #24914, #82561 ) ;
#62046=CIRCLE ( 'NONE', #5570, 0.06509327318403745899 ) ;
#62047=ORIENTED_EDGE ( 'NONE', *, *, #25565, .F. ) ;
#62048=DIRECTION ( 'NONE',  ( 0.000000000000000000, -0.000000000000000000, 1.000000000000000000 ) ) ;
#62049=LINE ( 'NONE', #101965, #70317 ) ;
#62050=FACE_OUTER_BOUND ( 'NONE', #82098, .T. ) ;
#62051=EDGE_LOOP ( 'NONE', ( #48428, #21, #102318, #58236 ) ) ;
#62052=EDGE_LOOP ( 'NONE', ( #55688, #83391, #44234, #116011 ) ) ;
#62053=EDGE_LOOP ( 'NONE', ( #101859, #99314, #89812, #102316 ) ) ;
#62054=AXIS2_PLACEMENT_3D ( 'NONE', #53799, #114021, #24352 ) ;
#62056=VECTOR ( 'NONE', #111316, 1000.000000000000000 ) ;
#62057=AXIS2_PLACEMENT_3D ( 'NONE', #47817, #108651, #27493 ) ;
#62058=ORIENTED_EDGE ( 'NONE', *, *, #98017, .T. ) ;
#62059=CARTESIAN_POINT ( 'NONE',  ( 1.449999999999952660, 2.500000000000000000, -6.841600689897078702 ) ) ;
#62060=DIRECTION ( 'NONE',  ( 0.000000000000000000, 0.000000000000000000, 1.000000000000000000 ) ) ;
#62061=VECTOR ( 'NONE', #113502, 1000.000000000000000 ) ;
#62062=DIRECTION ( 'NONE',  ( 0.000000000000000000, 0.000000000000000000, 1.000000000000000000 ) ) ;
#62063=ORIENTED_EDGE ( 'NONE', *, *, #18954, .F. ) ;
#62064=DIRECTION ( 'NONE',  ( -4.274815082592931898E-19, -0.9999939076577903929, -0.003490651415223739937 ) ) ;
#62066=DIRECTION ( 'NONE',  ( -0.000000000000000000, 1.000000000000000000, -0.000000000000000000 ) ) ;
#62067=FACE_OUTER_BOUND ( 'NONE', #40949, .T. ) ;
#62068=EDGE_CURVE ( 'NONE', #125864, #12245, #28817, .T. ) ;
#62069=DIRECTION ( 'NONE',  ( 0.000000000000000000, 0.000000000000000000, -1.000000000000000000 ) ) ;
#62070=ORIENTED_EDGE ( 'NONE', *, *, #80662, .F. ) ;
#62071=DIRECTION ( 'NONE',  ( 0.000000000000000000, 0.000000000000000000, 1.000000000000000000 ) ) ;
#62072=VERTEX_POINT ( 'NONE', #95176 ) ;
#62073=ORIENTED_EDGE ( 'NONE', *, *, #25073, .F. ) ;
#62075=CARTESIAN_POINT ( 'NONE',  ( -6.250000000000015987, 2.500000000000000000, 1.472243186433545459 ) ) ;
#62076=CIRCLE ( 'NONE', #18132, 0.09999999999999982514 ) ;
#62077=DIRECTION ( 'NONE',  ( -0.000000000000000000, 1.000000000000000000, -0.000000000000000000 ) ) ;
#62078=AXIS2_PLACEMENT_3D ( 'NONE', #92434, #42057, #83275 ) ;
#62079=DIRECTION ( 'NONE',  ( 0.000000000000000000, 0.000000000000000000, 1.000000000000000000 ) ) ;
#62080=AXIS2_PLACEMENT_3D ( 'NONE', #17729, #47866, #87759 ) ;
#62081=CARTESIAN_POINT ( 'NONE',  ( 87.50000000000001421, -3.975344334345451980, 6.360552532166690476 ) ) ;
#62082=CARTESIAN_POINT ( 'NONE',  ( 11.64999999999990443, 12.50000000000000000, 2.922977105672686982 ) ) ;
#62083=CONICAL_SURFACE ( 'NONE', #85039, 0.09999999999999999167, 0.003490658503988666988 ) ;
#62084=EDGE_CURVE ( 'NONE', #1556, #28294, #112443, .T. ) ;
#62085=DIRECTION ( 'NONE',  ( -0.000000000000000000, -1.000000000000000000, -0.000000000000000000 ) ) ;
#62086=DIRECTION ( 'NONE',  ( 0.000000000000000000, 0.000000000000000000, 1.000000000000000000 ) ) ;
#62087=AXIS2_PLACEMENT_3D ( 'NONE', #76332, #115586, #56028 ) ;
#62088=AXIS2_PLACEMENT_3D ( 'NONE', #71168, #88878, #128841 ) ;
#62089=FACE_OUTER_BOUND ( 'NONE', #35538, .T. ) ;
#62090=ORIENTED_EDGE ( 'NONE', *, *, #100077, .F. ) ;
#62091=VERTEX_POINT ( 'NONE', #26441 ) ;
#62092=AXIS2_PLACEMENT_3D ( 'NONE', #79967, #19768, #72096 ) ;
#62093=ORIENTED_EDGE ( 'NONE', *, *, #39273, .T. ) ;
#62094=ORIENTED_EDGE ( 'NONE', *, *, #62798, .T. ) ;
#62095=AXIS2_PLACEMENT_3D ( 'NONE', #45137, #15641, #16912 ) ;
#62096=ADVANCED_FACE ( 'NONE', ( #24501 ), #116626, .T. ) ;
#62097=CARTESIAN_POINT ( 'NONE',  ( -1.050000000000038680, 2.500000000000000000, 2.511473670974873507 ) ) ;
#62098=DIRECTION ( 'NONE',  ( 0.000000000000000000, 0.000000000000000000, 1.000000000000000000 ) ) ;
#62099=AXIS2_PLACEMENT_3D ( 'NONE', #102226, #123152, #72760 ) ;
#62100=ORIENTED_EDGE ( 'NONE', *, *, #38862, .T. ) ;
#62101=DIRECTION ( 'NONE',  ( 0.000000000000000000, 0.000000000000000000, 1.000000000000000000 ) ) ;
#62102=CIRCLE ( 'NONE', #36962, 0.1000000000000000472 ) ;
#62103=CIRCLE ( 'NONE', #5631, 0.09999999999999982514 ) ;
#62104=CARTESIAN_POINT ( 'NONE',  ( -7.499999999999976907, 2.500000000000000000, 4.330127018922196314 ) ) ;
#62105=VERTEX_POINT ( 'NONE', #5484 ) ;
#62106=EDGE_CURVE ( 'NONE', #66127, #33429, #18135, .T. ) ;
#62107=CARTESIAN_POINT ( 'NONE',  ( -10.00000000000000355, 12.50000000000000000, 3.637306695894644726 ) ) ;
#62108=DIRECTION ( 'NONE',  ( 0.000000000000000000, 0.000000000000000000, -1.000000000000000000 ) ) ;
#62109=VERTEX_POINT ( 'NONE', #84051 ) ;
#62110=EDGE_LOOP ( 'NONE', ( #119279, #97987 ) ) ;
#62111=VERTEX_POINT ( 'NONE', #93891 ) ;
#62112=ORIENTED_EDGE ( 'NONE', *, *, #16190, .F. ) ;
#62113=DIRECTION ( 'NONE',  ( 0.000000000000000000, 0.000000000000000000, -1.000000000000000000 ) ) ;
#62114=VECTOR ( 'NONE', #39183, 1000.000000000000000 ) ;
#62115=CARTESIAN_POINT ( 'NONE',  ( 4.999999999999933387, 12.50000000000000000, 5.022947341949748790 ) ) ;
#62116=DIRECTION ( 'NONE',  ( -4.274815082592931898E-19, -0.9999939076577903929, -0.003490651415223739937 ) ) ;
#62117=CARTESIAN_POINT ( 'NONE',  ( -0.4000000000000396572, 12.50000000000000000, 3.637306695894644726 ) ) ;
#62118=ORIENTED_EDGE ( 'NONE', *, *, #98325, .F. ) ;
#62119=EDGE_CURVE ( 'NONE', #35293, #63751, #110370, .T. ) ;
#62121=ORIENTED_EDGE ( 'NONE', *, *, #10106, .F. ) ;
#62122=CARTESIAN_POINT ( 'NONE',  ( -6.900000000000015454, 2.500000000000000000, 4.083716857408420609 ) ) ;
#62123=CARTESIAN_POINT ( 'NONE',  ( 2.500000000000002220, -2.499999999999999556, -9.999999999999998224 ) ) ;
#62124=CARTESIAN_POINT ( 'NONE',  ( -8.350000000000013856, 12.50000000000000000, -6.495190528383297135 ) ) ;
#62125=DIRECTION ( 'NONE',  ( -0.000000000000000000, -1.000000000000000000, -0.000000000000000000 ) ) ;
#62126=EDGE_CURVE ( 'NONE', #35145, #26812, #25783, .T. ) ;
#62127=EDGE_LOOP ( 'NONE', ( #117190, #68103 ) ) ;
#62129=AXIS2_PLACEMENT_3D ( 'NONE', #97189, #43761, #44378 ) ;
#62130=VERTEX_POINT ( 'NONE', #64419 ) ;
#62131=VERTEX_POINT ( 'NONE', #14657 ) ;
#62132=DIRECTION ( 'NONE',  ( 0.000000000000000000, 1.000000000000000000, 0.000000000000000000 ) ) ;
#62133=LINE ( 'NONE', #41851, #37284 ) ;
#62134=EDGE_CURVE ( 'NONE', #68530, #56898, #11874, .T. ) ;
#62135=ADVANCED_FACE ( 'NONE', ( #96443 ), #120840, .T. ) ;
#62136=DIRECTION ( 'NONE',  ( -0.000000000000000000, 1.000000000000000000, -0.000000000000000000 ) ) ;
#62137=EDGE_CURVE ( 'NONE', #80208, #118649, #34898, .T. ) ;
#62138=FACE_BOUND ( 'NONE', #10761, .T. ) ;
#62139=EDGE_CURVE ( 'NONE', #65087, #85338, #106282, .T. ) ;
#62140=FACE_OUTER_BOUND ( 'NONE', #49103, .T. ) ;
#62141=DIRECTION ( 'NONE',  ( 0.000000000000000000, 1.000000000000000000, 0.000000000000000000 ) ) ;
#62142=AXIS2_PLACEMENT_3D ( 'NONE', #96863, #77864, #55656 ) ;
#62143=CONICAL_SURFACE ( 'NONE', #72601, 0.1000000000000002554, 0.003490658503988666988 ) ;
#62144=CARTESIAN_POINT ( 'NONE',  ( -4.350000000000023626, 2.500000000000000000, 1.818653347947321475 ) ) ;
#62145=EDGE_CURVE ( 'NONE', #3135, #39693, #30693, .T. ) ;
#62146=DIRECTION ( 'NONE',  ( 0.000000000000000000, 0.000000000000000000, -1.000000000000000000 ) ) ;
#62147=EDGE_CURVE ( 'NONE', #42231, #25321, #91307, .T. ) ;
#62148=CARTESIAN_POINT ( 'NONE',  ( 8.349999999999919709, 2.500000000000000000, -1.472243186433550122 ) ) ;
#62149=ADVANCED_FACE ( 'NONE', ( #36909 ), #103835, .T. ) ;
#62150=DIRECTION ( 'NONE',  ( 0.000000000000000000, 1.000000000000000000, 0.000000000000000000 ) ) ;
#62151=ORIENTED_EDGE ( 'NONE', *, *, #66381, .T. ) ;
#62152=AXIS2_PLACEMENT_3D ( 'NONE', #43804, #64705, #64068 ) ;
#62153=CARTESIAN_POINT ( 'NONE',  ( -10.40000000000000213, 2.500000000000000000, 5.022947341949748790 ) ) ;
#62154=EDGE_CURVE ( 'NONE', #126358, #16718, #99917, .T. ) ;
#62155=AXIS2_PLACEMENT_3D ( 'NONE', #119955, #59772, #62332 ) ;
#62156=EDGE_CURVE ( 'NONE', #116689, #85338, #116334, .T. ) ;
#62157=CARTESIAN_POINT ( 'NONE',  ( -3.642919299551294898E-14, 2.500000000000000000, 0.6928203230275518099 ) ) ;
#62158=ORIENTED_EDGE ( 'NONE', *, *, #46584, .F. ) ;
#62159=ORIENTED_EDGE ( 'NONE', *, *, #97466, .T. ) ;
#62160=DIRECTION ( 'NONE',  ( 0.000000000000000000, 0.000000000000000000, 1.000000000000000000 ) ) ;
#62161=DIRECTION ( 'NONE',  ( 0.000000000000000000, -0.9999939076577903929, 0.003490651415223739937 ) ) ;
#62162=FACE_BOUND ( 'NONE', #125779, .T. ) ;
#62163=ADVANCED_FACE ( 'NONE', ( #46719 ), #26748, .T. ) ;
#62164=DIRECTION ( 'NONE',  ( 0.000000000000000000, 0.000000000000000000, -1.000000000000000000 ) ) ;
#62165=VERTEX_POINT ( 'NONE', #76828 ) ;
#62166=CARTESIAN_POINT ( 'NONE',  ( 0.000000000000000000, 2.500000000000000000, 0.1000000000000000056 ) ) ;
#62167=DIRECTION ( 'NONE',  ( 0.000000000000000000, 0.000000000000000000, 1.000000000000000000 ) ) ;
#62168=VECTOR ( 'NONE', #28865, 1000.000000000000000 ) ;
#62169=VERTEX_POINT ( 'NONE', #4839 ) ;
#62170=LINE ( 'NONE', #90971, #105507 ) ;
#62171=AXIS2_PLACEMENT_3D ( 'NONE', #77713, #69179, #60047 ) ;
#62172=CARTESIAN_POINT ( 'NONE',  ( -4.350000000000023626, 12.50000000000000000, 6.083687093685483660 ) ) ;
#62173=AXIS2_PLACEMENT_3D ( 'NONE', #13309, #12025, #53259 ) ;
#62174=VERTEX_POINT ( 'NONE', #44797 ) ;
#62175=DIRECTION ( 'NONE',  ( 0.000000000000000000, -0.000000000000000000, 1.000000000000000000 ) ) ;
#62176=CARTESIAN_POINT ( 'NONE',  ( 4.549999999999939426, 2.500000000000000000, -2.265063509461101798 ) ) ;
#62177=CIRCLE ( 'NONE', #99828, 0.06509327318403745899 ) ;
#62178=CONICAL_SURFACE ( 'NONE', #26570, 0.1000000000000000056, 0.003490658503988666988 ) ;
#62179=EDGE_LOOP ( 'NONE', ( #67813, #77011 ) ) ;
#62180=AXIS2_PLACEMENT_3D ( 'NONE', #11352, #51300, #110202 ) ;
#62181=CIRCLE ( 'NONE', #122807, 0.1000000000000002554 ) ;
#62182=LINE ( 'NONE', #11768, #71761 ) ;
#62183=CARTESIAN_POINT ( 'NONE',  ( -3.950000000000025491, 2.500000000000000000, 6.048780366869521252 ) ) ;
#62184=CARTESIAN_POINT ( 'NONE',  ( 6.249999999999967137, 2.500000000000000000, 6.595190528383296780 ) ) ;
#62185=VERTEX_POINT ( 'NONE', #34988 ) ;
#62186=EDGE_LOOP ( 'NONE', ( #34785, #9102, #6627, #101554 ) ) ;
#62187=CONICAL_SURFACE ( 'NONE', #122812, 0.1000000000000002554, 0.003490658503988666988 ) ;
#62188=DIRECTION ( 'NONE',  ( 0.000000000000000000, 1.000000000000000000, 0.000000000000000000 ) ) ;
#62189=VERTEX_POINT ( 'NONE', #114802 ) ;
#62190=CARTESIAN_POINT ( 'NONE',  ( -3.550000000000027356, 2.500000000000000000, 1.818653347947321475 ) ) ;
#62191=DIRECTION ( 'NONE',  ( 0.000000000000000000, 0.000000000000000000, -1.000000000000000000 ) ) ;
#62192=ADVANCED_FACE ( 'NONE', ( #128532 ), #85035, .T. ) ;
#62193=CONICAL_SURFACE ( 'NONE', #5722, 0.1000000000000002554, 0.003490658503988666988 ) ;
#62194=VECTOR ( 'NONE', #22108, 1000.000000000000000 ) ;
#62195=DIRECTION ( 'NONE',  ( -0.000000000000000000, 1.000000000000000000, -0.000000000000000000 ) ) ;
#62196=ORIENTED_EDGE ( 'NONE', *, *, #51964, .F. ) ;
#62197=FACE_OUTER_BOUND ( 'NONE', #60240, .T. ) ;
#62198=EDGE_CURVE ( 'NONE', #77843, #48167, #76924, .T. ) ;
#62199=CARTESIAN_POINT ( 'NONE',  ( 2.899999999999946620, 2.500000000000000000, -3.537306695894649966 ) ) ;
#62200=DIRECTION ( 'NONE',  ( -0.000000000000000000, 1.000000000000000000, -0.000000000000000000 ) ) ;
#62201=CARTESIAN_POINT ( 'NONE',  ( -6.050000000000018474, 2.500000000000000000, 6.841600689897072485 ) ) ;
#62202=DIRECTION ( 'NONE',  ( 0.000000000000000000, -0.000000000000000000, 1.000000000000000000 ) ) ;
#62203=DIRECTION ( 'NONE',  ( 0.000000000000000000, 0.000000000000000000, 1.000000000000000000 ) ) ;
#62204=EDGE_CURVE ( 'NONE', #21147, #107141, #9373, .T. ) ;
#62205=ORIENTED_EDGE ( 'NONE', *, *, #35527, .F. ) ;
#62206=ORIENTED_EDGE ( 'NONE', *, *, #73606, .T. ) ;
#62207=DIRECTION ( 'NONE',  ( 0.000000000000000000, 0.000000000000000000, 1.000000000000000000 ) ) ;
#62208=EDGE_LOOP ( 'NONE', ( #79427, #15626 ) ) ;
#62209=CARTESIAN_POINT ( 'NONE',  ( -4.600000000000028066, 2.500000000000000000, -5.122947341949753763 ) ) ;
#62210=EDGE_LOOP ( 'NONE', ( #79561, #9964, #54588, #113106 ) ) ;
#62211=ORIENTED_EDGE ( 'NONE', *, *, #114279, .F. ) ;
#62212=EDGE_LOOP ( 'NONE', ( #10745, #66791, #18458, #11480 ) ) ;
#62213=AXIS2_PLACEMENT_3D ( 'NONE', #116684, #57783, #76127 ) ;
#62214=LINE ( 'NONE', #102124, #45671 ) ;
#62215=DIRECTION ( 'NONE',  ( 0.000000000000000000, 0.000000000000000000, -1.000000000000000000 ) ) ;
#62216=CARTESIAN_POINT ( 'NONE',  ( -3.350000000000028511, 2.500000000000000000, 1.472243186433545459 ) ) ;
#62217=DIRECTION ( 'NONE',  ( 0.000000000000000000, 1.000000000000000000, 0.000000000000000000 ) ) ;
#62218=DIRECTION ( 'NONE',  ( 0.000000000000000000, 0.000000000000000000, -1.000000000000000000 ) ) ;
#62219=CARTESIAN_POINT ( 'NONE',  ( 1.649999999999950617, 12.50000000000000000, 2.165063509461097713 ) ) ;
#62220=DIRECTION ( 'NONE',  ( -0.000000000000000000, 1.000000000000000000, -0.000000000000000000 ) ) ;
#62221=DIRECTION ( 'NONE',  ( 0.000000000000000000, 0.000000000000000000, 1.000000000000000000 ) ) ;
#62223=CIRCLE ( 'NONE', #93510, 0.06509327318403745899 ) ;
#62224=ORIENTED_EDGE ( 'NONE', *, *, #96213, .F. ) ;
#62225=LINE ( 'NONE', #110660, #107134 ) ;
#62226=ORIENTED_EDGE ( 'NONE', *, *, #128982, .F. ) ;
#62227=EDGE_LOOP ( 'NONE', ( #100015, #20446, #46802, #100315 ) ) ;
#62228=CARTESIAN_POINT ( 'NONE',  ( -8.750000000000005329, 2.500000000000000000, 5.802370205355744659 ) ) ;
#62229=CARTESIAN_POINT ( 'NONE',  ( 10.59999999999990905, 2.500000000000000000, -4.576537180435978236 ) ) ;
#62230=LINE ( 'NONE', #111973, #23556 ) ;
#62231=AXIS2_PLACEMENT_3D ( 'NONE', #60043, #119570, #99949 ) ;
#62232=ADVANCED_FACE ( 'NONE', ( #38867 ), #37226, .T. ) ;
#62233=DIRECTION ( 'NONE',  ( 0.000000000000000000, 1.000000000000000000, 0.000000000000000000 ) ) ;
#62234=CIRCLE ( 'NONE', #35054, 0.06509327318403741736 ) ;
#62235=AXIS2_PLACEMENT_3D ( 'NONE', #97753, #98384, #127232 ) ;
#62236=FACE_OUTER_BOUND ( 'NONE', #87564, .T. ) ;
#62237=DIRECTION ( 'NONE',  ( 0.000000000000000000, -0.000000000000000000, 1.000000000000000000 ) ) ;
#62238=PLANE ( 'NONE',  #65605 ) ;
#62240=EDGE_LOOP ( 'NONE', ( #103468, #80156 ) ) ;
#62241=VECTOR ( 'NONE', #90979, 1000.000000000000000 ) ;
#62242=VERTEX_POINT ( 'NONE', #129175 ) ;
#62243=ORIENTED_EDGE ( 'NONE', *, *, #93773, .F. ) ;
#62244=EDGE_CURVE ( 'NONE', #35299, #14887, #57836, .T. ) ;
#62245=CIRCLE ( 'NONE', #72701, 0.1000000000000000472 ) ;
#62246=EDGE_CURVE ( 'NONE', #74354, #115572, #93368, .T. ) ;
#62247=ORIENTED_EDGE ( 'NONE', *, *, #70691, .T. ) ;
#62248=DIRECTION ( 'NONE',  ( 0.000000000000000000, 0.000000000000000000, 1.000000000000000000 ) ) ;
#62249=FACE_OUTER_BOUND ( 'NONE', #679, .T. ) ;
#62250=CIRCLE ( 'NONE', #81122, 0.06509327318403745899 ) ;
#62251=DIRECTION ( 'NONE',  ( 0.000000000000000000, 0.000000000000000000, 1.000000000000000000 ) ) ;
#62252=DIRECTION ( 'NONE',  ( -0.000000000000000000, -1.000000000000000000, -0.000000000000000000 ) ) ;
#62253=CIRCLE ( 'NONE', #87269, 0.09999999999999982514 ) ;
#62254=DIRECTION ( 'NONE',  ( 0.000000000000000000, 0.000000000000000000, 1.000000000000000000 ) ) ;
#62255=VERTEX_POINT ( 'NONE', #49965 ) ;
#62256=DIRECTION ( 'NONE',  ( 0.000000000000000000, 1.000000000000000000, 0.000000000000000000 ) ) ;
#62257=CARTESIAN_POINT ( 'NONE',  ( 0.6499999999999566125, 12.50000000000000000, -6.841600689897077814 ) ) ;
#62258=EDGE_CURVE ( 'NONE', #113976, #108759, #30321, .T. ) ;
#62259=DIRECTION ( 'NONE',  ( 0.000000000000000000, 1.000000000000000000, 0.000000000000000000 ) ) ;
#62260=PLANE ( 'NONE',  #20082 ) ;
#62261=CIRCLE ( 'NONE', #41339, 0.09999999999999982514 ) ;
#62262=AXIS2_PLACEMENT_3D ( 'NONE', #119573, #127483, #28642 ) ;
#62263=CARTESIAN_POINT ( 'NONE',  ( -7.950000000000012612, 2.500000000000000000, -2.165063509461101710 ) ) ;
#62264=ORIENTED_EDGE ( 'NONE', *, *, #2582, .F. ) ;
#62265=CIRCLE ( 'NONE', #87364, 0.09999999999999982514 ) ;
#62266=ORIENTED_EDGE ( 'NONE', *, *, #18080, .F. ) ;
#62267=ORIENTED_EDGE ( 'NONE', *, *, #50132, .F. ) ;
#62268=DIRECTION ( 'NONE',  ( 0.000000000000000000, 0.000000000000000000, -1.000000000000000000 ) ) ;
#62269=VERTEX_POINT ( 'NONE', #29658 ) ;
#62270=CARTESIAN_POINT ( 'NONE',  ( 9.399999999999915090, 2.500000000000000000, 4.676537180435972552 ) ) ;
#62271=DIRECTION ( 'NONE',  ( 0.000000000000000000, 0.000000000000000000, 1.000000000000000000 ) ) ;
#62272=AXIS2_PLACEMENT_3D ( 'NONE', #50355, #90258, #90927 ) ;
#62273=ORIENTED_EDGE ( 'NONE', *, *, #114910, .F. ) ;
#62274=LINE ( 'NONE', #72730, #43272 ) ;
#62275=CARTESIAN_POINT ( 'NONE',  ( -13.54999999999999005, 2.500000000000000000, 2.411473670974877415 ) ) ;
#62276=AXIS2_PLACEMENT_3D ( 'NONE', #9563, #48854, #99238 ) ;
#62277=CARTESIAN_POINT ( 'NONE',  ( -0.8500000000000382805, 2.500000000000000000, -1.472243186433550122 ) ) ;
#62278=DIRECTION ( 'NONE',  ( 0.000000000000000000, 1.000000000000000000, 0.000000000000000000 ) ) ;
#62279=EDGE_CURVE ( 'NONE', #76856, #44317, #27708, .T. ) ;
#62281=VECTOR ( 'NONE', #109676, 1000.000000000000000 ) ;
#62282=LINE ( 'NONE', #110082, #16344 ) ;
#62283=EDGE_LOOP ( 'NONE', ( #96744, #27088 ) ) ;
#62284=ORIENTED_EDGE ( 'NONE', *, *, #60380, .F. ) ;
#62285=EDGE_CURVE ( 'NONE', #103089, #124700, #66163, .T. ) ;
#62287=LINE ( 'NONE', #101559, #7971 ) ;
#62288=EDGE_CURVE ( 'NONE', #118069, #125289, #70659, .T. ) ;
#62289=CARTESIAN_POINT ( 'NONE',  ( 6.899999999999926636, 2.500000000000000000, 0.2464101615137736789 ) ) ;
#62290=CARTESIAN_POINT ( 'NONE',  ( 3.299999999999944755, 2.500000000000000000, -2.385244779468109755E-15 ) ) ;
#62291=ORIENTED_EDGE ( 'NONE', *, *, #94664, .T. ) ;
#62292=EDGE_CURVE ( 'NONE', #54553, #128976, #57870, .T. ) ;
#62293=EDGE_CURVE ( 'NONE', #109985, #9468, #110087, .T. ) ;
#62294=EDGE_LOOP ( 'NONE', ( #38280, #108540, #26447, #21226 ) ) ;
#62295=DIRECTION ( 'NONE',  ( -0.000000000000000000, -1.000000000000000000, -0.000000000000000000 ) ) ;
#62296=DIRECTION ( 'NONE',  ( -0.000000000000000000, -1.000000000000000000, -0.000000000000000000 ) ) ;
#62297=EDGE_CURVE ( 'NONE', #2356, #3164, #87372, .T. ) ;
#62298=CARTESIAN_POINT ( 'NONE',  ( 5.399999999999934630, 12.50000000000000000, 0.6928203230275494784 ) ) ;
#62299=CARTESIAN_POINT ( 'NONE',  ( -1.450000000000035483, 2.500000000000000000, 6.148780366869520897 ) ) ;
#62300=EDGE_LOOP ( 'NONE', ( #109905, #61537, #21763, #38476 ) ) ;
#62301=CARTESIAN_POINT ( 'NONE',  ( 1.249999999999954259, 12.50000000000000000, -7.188010851410854052 ) ) ;
#62302=ADVANCED_FACE ( 'NONE', ( #87273 ), #9743, .T. ) ;
#62303=DIRECTION ( 'NONE',  ( 0.000000000000000000, 0.000000000000000000, 1.000000000000000000 ) ) ;
#62304=VERTEX_POINT ( 'NONE', #19164 ) ;
#62305=VECTOR ( 'NONE', #124798, 1000.000000000000000 ) ;
#62306=FACE_OUTER_BOUND ( 'NONE', #123508, .T. ) ;
#62307=ORIENTED_EDGE ( 'NONE', *, *, #17046, .T. ) ;
#62308=EDGE_CURVE ( 'NONE', #90957, #70171, #80044, .T. ) ;
#62309=PLANE ( 'NONE',  #116450 ) ;
#62310=AXIS2_PLACEMENT_3D ( 'NONE', #51276, #52543, #11964 ) ;
#62311=VECTOR ( 'NONE', #100264, 1000.000000000000000 ) ;
#62312=ORIENTED_EDGE ( 'NONE', *, *, #67373, .T. ) ;
#62313=CARTESIAN_POINT ( 'NONE',  ( -4.150000000000027889, 2.500000000000000000, -6.595190528383302109 ) ) ;
#62314=DIRECTION ( 'NONE',  ( -0.000000000000000000, -1.000000000000000000, -0.000000000000000000 ) ) ;
#62315=EDGE_LOOP ( 'NONE', ( #105320, #56670, #33215, #80030 ) ) ;
#62316=ORIENTED_EDGE ( 'NONE', *, *, #38797, .T. ) ;
#62319=CARTESIAN_POINT ( 'NONE',  ( -6.250000000000015987, 2.500000000000000000, 1.572243186433545548 ) ) ;
#62321=AXIS2_PLACEMENT_3D ( 'NONE', #53701, #93631, #81237 ) ;
#62322=DIRECTION ( 'NONE',  ( 0.000000000000000000, 1.000000000000000000, 0.000000000000000000 ) ) ;
#62323=CARTESIAN_POINT ( 'NONE',  ( -0.4000000000000401013, 2.500000000000000000, -3.637306695894650055 ) ) ;
#62324=DIRECTION ( 'NONE',  ( -0.000000000000000000, -1.000000000000000000, -0.000000000000000000 ) ) ;
#62325=DIRECTION ( 'NONE',  ( -0.000000000000000000, -1.000000000000000000, -0.000000000000000000 ) ) ;
#62326=DIRECTION ( 'NONE',  ( -4.274815082592931898E-19, -0.9999939076577903929, -0.003490651415223739937 ) ) ;
#62327=CIRCLE ( 'NONE', #22630, 0.06509327318403745899 ) ;
#62328=EDGE_LOOP ( 'NONE', ( #9361, #22450, #104996, #83043 ) ) ;
#62329=EDGE_LOOP ( 'NONE', ( #117064, #108163, #62751, #91223 ) ) ;
#62330=CARTESIAN_POINT ( 'NONE',  ( 8.149999999999920419, 2.500000000000000000, -1.818653347947325916 ) ) ;
#62331=ORIENTED_EDGE ( 'NONE', *, *, #6500, .T. ) ;
#62332=DIRECTION ( 'NONE',  ( 0.000000000000000000, -0.000000000000000000, 1.000000000000000000 ) ) ;
#62333=FACE_OUTER_BOUND ( 'NONE', #64605, .T. ) ;
#62334=CONICAL_SURFACE ( 'NONE', #106149, 0.1000000000000002554, 0.003490658503988666988 ) ;
#62335=PLANE ( 'NONE',  #3065 ) ;
#62336=VERTEX_POINT ( 'NONE', #37554 ) ;
#62337=ORIENTED_EDGE ( 'NONE', *, *, #77041, .T. ) ;
#62338=FACE_BOUND ( 'NONE', #30976, .T. ) ;
#62339=ORIENTED_EDGE ( 'NONE', *, *, #56009, .T. ) ;
#62340=CARTESIAN_POINT ( 'NONE',  ( -2.499999999999996003, 12.50000000000000000, 0.06509327318403515528 ) ) ;
#62341=DIRECTION ( 'NONE',  ( -0.000000000000000000, -1.000000000000000000, -0.000000000000000000 ) ) ;
#62342=DIRECTION ( 'NONE',  ( 0.000000000000000000, 0.000000000000000000, 1.000000000000000000 ) ) ;
#62343=VECTOR ( 'NONE', #102626, 1000.000000000000000 ) ;
#62344=DIRECTION ( 'NONE',  ( 0.000000000000000000, 1.000000000000000000, 0.000000000000000000 ) ) ;
#62345=ADVANCED_FACE ( 'NONE', ( #127852 ), #99044, .T. ) ;
#62346=LINE ( 'NONE', #100331, #82679 ) ;
#62347=CARTESIAN_POINT ( 'NONE',  ( -13.29999999999999005, 2.500000000000000000, -4.330127018922198978 ) ) ;
#62348=DIRECTION ( 'NONE',  ( 0.000000000000000000, 0.000000000000000000, -1.000000000000000000 ) ) ;
#62349=DIRECTION ( 'NONE',  ( -0.000000000000000000, 1.000000000000000000, -0.000000000000000000 ) ) ;
#62350=CARTESIAN_POINT ( 'NONE',  ( 10.84999999999990905, 2.500000000000000000, -5.802370205355749988 ) ) ;
#62351=CARTESIAN_POINT ( 'NONE',  ( -4.076600168545496672E-14, 2.500000000000000000, -4.922947341949753586 ) ) ;
#62352=AXIS2_PLACEMENT_3D ( 'NONE', #113381, #121925, #102915 ) ;
#62353=AXIS2_PLACEMENT_3D ( 'NONE', #81825, #92292, #53666 ) ;
#62354=CARTESIAN_POINT ( 'NONE',  ( -1.250000000000001554, 12.50000000000000000, 6.495190528383297135 ) ) ;
#62355=EDGE_CURVE ( 'NONE', #2098, #51142, #82911, .T. ) ;
#62357=AXIS2_PLACEMENT_3D ( 'NONE', #101551, #110710, #100887 ) ;
#62358=ORIENTED_EDGE ( 'NONE', *, *, #76516, .T. ) ;
#62359=VERTEX_POINT ( 'NONE', #18541 ) ;
#62360=DIRECTION ( 'NONE',  ( 0.000000000000000000, 0.000000000000000000, 1.000000000000000000 ) ) ;
#62361=VERTEX_POINT ( 'NONE', #58493 ) ;
#62362=DIRECTION ( 'NONE',  ( -4.274815082592931898E-19, -0.9999939076577903929, -0.003490651415223739937 ) ) ;
#62363=PLANE ( 'NONE',  #31990 ) ;
#62364=ORIENTED_EDGE ( 'NONE', *, *, #10416, .F. ) ;
#62365=EDGE_LOOP ( 'NONE', ( #63350, #28789 ) ) ;
#62366=AXIS2_PLACEMENT_3D ( 'NONE', #2764, #32896, #63633 ) ;
#62367=ORIENTED_EDGE ( 'NONE', *, *, #30077, .T. ) ;
#62368=CARTESIAN_POINT ( 'NONE',  ( -13.09999999999999254, 12.50000000000000000, -0.3464101615137741286 ) ) ;
#62369=PLANE ( 'NONE',  #27948 ) ;
#62370=DIRECTION ( 'NONE',  ( 0.000000000000000000, 1.000000000000000000, 0.000000000000000000 ) ) ;
#62371=CARTESIAN_POINT ( 'NONE',  ( -9.150000000000005684, 2.500000000000000000, 5.802370205355744659 ) ) ;
#62372=FACE_OUTER_BOUND ( 'NONE', #105050, .T. ) ;
#62373=CARTESIAN_POINT ( 'NONE',  ( -2.300000000000033573, 12.50000000000000000, -4.048810130592463530 ) ) ;
#62374=VECTOR ( 'NONE', #43326, 1000.000000000000000 ) ;
#62375=VERTEX_POINT ( 'NONE', #48657 ) ;
#62376=CARTESIAN_POINT ( 'NONE',  ( -7.300000000000014921, 12.50000000000000000, 4.741630453620009789 ) ) ;
#62377=ORIENTED_EDGE ( 'NONE', *, *, #85925, .T. ) ;
#62378=CIRCLE ( 'NONE', #16358, 0.1000000000000002554 ) ;
#62379=AXIS2_PLACEMENT_3D ( 'NONE', #91732, #123131, #92364 ) ;
#62380=VERTEX_POINT ( 'NONE', #40791 ) ;
#62381=VERTEX_POINT ( 'NONE', #80702 ) ;
#62382=CARTESIAN_POINT ( 'NONE',  ( -6.650000000000019007, 2.500000000000000000, -5.802370205355749988 ) ) ;
#62384=VERTEX_POINT ( 'NONE', #41431 ) ;
#62385=ORIENTED_EDGE ( 'NONE', *, *, #29183, .T. ) ;
#62386=EDGE_CURVE ( 'NONE', #4792, #121198, #24412, .T. ) ;
#62388=CARTESIAN_POINT ( 'NONE',  ( -5.000000000000023093, 12.50000000000000000, 0.6928203230275494784 ) ) ;
#62389=CARTESIAN_POINT ( 'NONE',  ( 7.049999999999928768, 2.500000000000000000, 6.595190528383296780 ) ) ;
#62390=CARTESIAN_POINT ( 'NONE',  ( 10.59999999999990905, 12.50000000000000000, 3.983716857408420076 ) ) ;
#62391=DIRECTION ( 'NONE',  ( 0.000000000000000000, 1.000000000000000000, 0.000000000000000000 ) ) ;
#62392=AXIS2_PLACEMENT_3D ( 'NONE', #82455, #122371, #53622 ) ;
#62393=FACE_OUTER_BOUND ( 'NONE', #2685, .T. ) ;
#62394=ADVANCED_FACE ( 'NONE', ( #43360 ), #45443, .T. ) ;
#62395=EDGE_LOOP ( 'NONE', ( #101044, #70027, #76927, #44006 ) ) ;
#62396=AXIS2_PLACEMENT_3D ( 'NONE', #122469, #22975, #63541 ) ;
#62397=DIRECTION ( 'NONE',  ( 0.000000000000000000, 1.000000000000000000, 0.000000000000000000 ) ) ;
#62398=AXIS2_PLACEMENT_3D ( 'NONE', #42934, #82846, #33106 ) ;
#62399=ORIENTED_EDGE ( 'NONE', *, *, #115326, .F. ) ;
#62400=FACE_OUTER_BOUND ( 'NONE', #69155, .T. ) ;
#62401=CONICAL_SURFACE ( 'NONE', #37266, 0.1000000000000000472, 0.003490658503988666988 ) ;
#62402=ORIENTED_EDGE ( 'NONE', *, *, #106786, .T. ) ;
#62403=DIRECTION ( 'NONE',  ( 0.000000000000000000, -0.000000000000000000, 1.000000000000000000 ) ) ;
#62404=ADVANCED_FACE ( 'NONE', ( #120615 ), #85128, .T. ) ;
#62405=EDGE_CURVE ( 'NONE', #61045, #79468, #93460, .T. ) ;
#62406=VERTEX_POINT ( 'NONE', #71505 ) ;
#62407=CIRCLE ( 'NONE', #10163, 0.1000000000000000472 ) ;
#62408=LINE ( 'NONE', #61765, #65256 ) ;
#62409=AXIS2_PLACEMENT_3D ( 'NONE', #71364, #90361, #72677 ) ;
#62410=AXIS2_PLACEMENT_3D ( 'NONE', #73787, #101334, #101975 ) ;
#62411=ADVANCED_FACE ( 'NONE', ( #121258 ), #87181, .T. ) ;
#62412=DIRECTION ( 'NONE',  ( 0.000000000000000000, 1.000000000000000000, 0.000000000000000000 ) ) ;
#62413=ORIENTED_EDGE ( 'NONE', *, *, #50023, .F. ) ;
#62414=ORIENTED_EDGE ( 'NONE', *, *, #67717, .F. ) ;
#62415=FACE_OUTER_BOUND ( 'NONE', #61475, .T. ) ;
#62416=CARTESIAN_POINT ( 'NONE',  ( 3.949999999999940670, 2.500000000000000000, 1.718653347947321386 ) ) ;
#62417=ADVANCED_FACE ( 'NONE', ( #73432 ), #66260, .T. ) ;
#62418=CARTESIAN_POINT ( 'NONE',  ( 4.599999999999935696, 2.500000000000000000, 5.022947341949748790 ) ) ;
#62419=CARTESIAN_POINT ( 'NONE',  ( -0.4000000000000392131, 2.500000000000000000, -4.922947341949753586 ) ) ;
#62420=VECTOR ( 'NONE', #18166, 1000.000000000000000 ) ;
#62421=FACE_OUTER_BOUND ( 'NONE', #114859, .T. ) ;
#62422=CIRCLE ( 'NONE', #70804, 0.1000000000000002554 ) ;
#62423=ORIENTED_EDGE ( 'NONE', *, *, #4481, .F. ) ;
#62424=CARTESIAN_POINT ( 'NONE',  ( 9.149999999999915090, 2.500000000000000000, -2.165063509461101710 ) ) ;
#62425=ORIENTED_EDGE ( 'NONE', *, *, #8310, .T. ) ;
#62426=CARTESIAN_POINT ( 'NONE',  ( -9.350000000000008527, 12.50000000000000000, -6.906693963081109722 ) ) ;
#62427=DIRECTION ( 'NONE',  ( 0.000000000000000000, 0.000000000000000000, 1.000000000000000000 ) ) ;
#62428=CIRCLE ( 'NONE', #93706, 0.1000000000000002554 ) ;
#62429=ADVANCED_FACE ( 'NONE', ( #11939 ), #108119, .T. ) ;
#62430=AXIS2_PLACEMENT_3D ( 'NONE', #76826, #28374, #8070 ) ;
#62431=VECTOR ( 'NONE', #56432, 1000.000000000000000 ) ;
#62432=DIRECTION ( 'NONE',  ( -0.000000000000000000, 1.000000000000000000, -0.000000000000000000 ) ) ;
#62433=DIRECTION ( 'NONE',  ( 0.000000000000000000, 0.000000000000000000, 1.000000000000000000 ) ) ;
#62434=DIRECTION ( 'NONE',  ( 0.000000000000000000, 1.000000000000000000, 0.000000000000000000 ) ) ;
#62435=DIRECTION ( 'NONE',  ( -0.000000000000000000, 1.000000000000000000, -0.000000000000000000 ) ) ;
#62437=ORIENTED_EDGE ( 'NONE', *, *, #106164, .T. ) ;
#62438=CARTESIAN_POINT ( 'NONE',  ( 3.299999999999944755, 2.500000000000000000, -4.330127018922201643 ) ) ;
#62439=EDGE_CURVE ( 'NONE', #22140, #27344, #112244, .T. ) ;
#62440=DIRECTION ( 'NONE',  ( 0.000000000000000000, -0.9999939076577903929, 0.003490651415223739937 ) ) ;
#62441=DIRECTION ( 'NONE',  ( 0.000000000000000000, -0.000000000000000000, 1.000000000000000000 ) ) ;
#62442=ORIENTED_EDGE ( 'NONE', *, *, #52939, .T. ) ;
#62443=ORIENTED_EDGE ( 'NONE', *, *, #8294, .F. ) ;
#62444=AXIS2_PLACEMENT_3D ( 'NONE', #110338, #20678, #50777 ) ;
#62445=EDGE_CURVE ( 'NONE', #49778, #26094, #14017, .T. ) ;
#62446=DIRECTION ( 'NONE',  ( 0.000000000000000000, 1.000000000000000000, 0.000000000000000000 ) ) ;
#62447=CIRCLE ( 'NONE', #104292, 0.06509327318403745899 ) ;
#62448=VERTEX_POINT ( 'NONE', #42059 ) ;
#62449=ORIENTED_EDGE ( 'NONE', *, *, #54661, .F. ) ;
#62450=DIRECTION ( 'NONE',  ( 0.000000000000000000, 1.000000000000000000, 0.000000000000000000 ) ) ;
#62451=EDGE_CURVE ( 'NONE', #63624, #93574, #110782, .T. ) ;
#62452=ORIENTED_EDGE ( 'NONE', *, *, #78735, .F. ) ;
#62453=CARTESIAN_POINT ( 'NONE',  ( 20.06694580393454785, -2.635910463901357303, -2.269534205241988456 ) ) ;
#62454=AXIS2_PLACEMENT_3D ( 'NONE', #37390, #115258, #87111 ) ;
#62455=DIRECTION ( 'NONE',  ( -0.000000000000000000, -1.000000000000000000, -0.000000000000000000 ) ) ;
#62456=ADVANCED_FACE ( 'NONE', ( #61709 ), #53175, .T. ) ;
#62457=CARTESIAN_POINT ( 'NONE',  ( 16.68526679984121586, 0.4774970013478979647, 5.954360761637129684 ) ) ;
#62458=EDGE_CURVE ( 'NONE', #125340, #3331, #32833, .T. ) ;
#62459=EDGE_LOOP ( 'NONE', ( #85258, #7808, #29762, #45050 ) ) ;
#62460=DIRECTION ( 'NONE',  ( 0.000000000000000000, 1.000000000000000000, 0.000000000000000000 ) ) ;
#62461=CIRCLE ( 'NONE', #110556, 0.06509327318403745899 ) ;
#62462=EDGE_CURVE ( 'NONE', #37733, #85672, #100335, .T. ) ;
#62463=DIRECTION ( 'NONE',  ( 0.000000000000000000, 0.000000000000000000, 1.000000000000000000 ) ) ;
#62464=CIRCLE ( 'NONE', #104304, 0.1000000000000000472 ) ;
#62465=ORIENTED_EDGE ( 'NONE', *, *, #88354, .F. ) ;
#62466=ADVANCED_FACE ( 'NONE', ( #122557 ), #72809, .T. ) ;
#62467=CIRCLE ( 'NONE', #112633, 0.06509327318403745899 ) ;
#62468=VECTOR ( 'NONE', #72579, 1000.000000000000000 ) ;
#62469=EDGE_CURVE ( 'NONE', #55655, #47265, #89252, .T. ) ;
#62470=ORIENTED_EDGE ( 'NONE', *, *, #92554, .F. ) ;
#62471=ORIENTED_EDGE ( 'NONE', *, *, #77809, .T. ) ;
#62472=CARTESIAN_POINT ( 'NONE',  ( -2.900000000000030109, 2.500000000000000000, -3.537306695894649966 ) ) ;
#62473=DIRECTION ( 'NONE',  ( 0.000000000000000000, 0.000000000000000000, 1.000000000000000000 ) ) ;
#62474=DIRECTION ( 'NONE',  ( 0.000000000000000000, 0.000000000000000000, 1.000000000000000000 ) ) ;
#62475=FACE_BOUND ( 'NONE', #108930, .T. ) ;
#62476=ORIENTED_EDGE ( 'NONE', *, *, #43414, .F. ) ;
#62477=PLANE ( 'NONE',  #4914 ) ;
#62478=DIRECTION ( 'NONE',  ( -0.000000000000000000, 1.000000000000000000, -0.000000000000000000 ) ) ;
#62479=ORIENTED_EDGE ( 'NONE', *, *, #18656, .F. ) ;
#62480=DIRECTION ( 'NONE',  ( 0.000000000000000000, 1.000000000000000000, 0.000000000000000000 ) ) ;
#62481=FACE_OUTER_BOUND ( 'NONE', #16896, .T. ) ;
#62483=CARTESIAN_POINT ( 'NONE',  ( 2.500000000000002220, -1.500000000000000000, 10.00000000000000178 ) ) ;
#62484=VECTOR ( 'NONE', #63122, 1000.000000000000000 ) ;
#62485=DIRECTION ( 'NONE',  ( 0.000000000000000000, 0.000000000000000000, 1.000000000000000000 ) ) ;
#62486=PLANE ( 'NONE',  #116160 ) ;
#62487=CARTESIAN_POINT ( 'NONE',  ( 3.749999999999942268, 2.500000000000000000, 1.472243186433545459 ) ) ;
#62489=AXIS2_PLACEMENT_3D ( 'NONE', #3308, #18598, #43253 ) ;
#62490=ORIENTED_EDGE ( 'NONE', *, *, #10660, .F. ) ;
#62491=EDGE_LOOP ( 'NONE', ( #36284, #109493, #103550, #77758 ) ) ;
#62492=AXIS2_PLACEMENT_3D ( 'NONE', #103261, #113063, #81676 ) ;
#62493=EDGE_LOOP ( 'NONE', ( #125464, #58674, #70131, #83537 ) ) ;
#62494=VERTEX_POINT ( 'NONE', #1471 ) ;
#62495=PLANE ( 'NONE',  #22354 ) ;
#62496=DIRECTION ( 'NONE',  ( 0.000000000000000000, 0.000000000000000000, -1.000000000000000000 ) ) ;
#62497=DIRECTION ( 'NONE',  ( 0.000000000000000000, -0.9999939076577903929, 0.003490651415223739937 ) ) ;
#62498=ORIENTED_EDGE ( 'NONE', *, *, #28908, .T. ) ;
#62499=FACE_BOUND ( 'NONE', #78051, .T. ) ;
#62500=DIRECTION ( 'NONE',  ( 0.000000000000000000, 1.000000000000000000, 0.000000000000000000 ) ) ;
#62501=DIRECTION ( 'NONE',  ( 0.000000000000000000, 0.000000000000000000, 1.000000000000000000 ) ) ;
#62502=AXIS2_PLACEMENT_3D ( 'NONE', #36971, #76893, #28443 ) ;
#62503=AXIS2_PLACEMENT_3D ( 'NONE', #55607, #115137, #75887 ) ;
#62504=PLANE ( 'NONE',  #72145 ) ;
#62505=AXIS2_PLACEMENT_3D ( 'NONE', #84902, #126114, #44327 ) ;
#62506=LINE ( 'NONE', #32414, #51185 ) ;
#62507=CARTESIAN_POINT ( 'NONE',  ( 5.849999999999933920, 12.50000000000000000, -2.857883832488653741 ) ) ;
#62508=CARTESIAN_POINT ( 'NONE',  ( -9.550000000000006040, 2.500000000000000000, 2.165063509461097713 ) ) ;
#62509=CARTESIAN_POINT ( 'NONE',  ( -5.850000000000018296, 2.500000000000000000, 5.902370205355745192 ) ) ;
#62510=DIRECTION ( 'NONE',  ( 0.000000000000000000, 1.000000000000000000, 0.000000000000000000 ) ) ;
#62511=DIRECTION ( 'NONE',  ( 0.000000000000000000, 1.000000000000000000, 0.000000000000000000 ) ) ;
#62512=AXIS2_PLACEMENT_3D ( 'NONE', #35100, #75011, #54079 ) ;
#62513=ORIENTED_EDGE ( 'NONE', *, *, #83683, .T. ) ;
#62514=EDGE_CURVE ( 'NONE', #108066, #121486, #111418, .T. ) ;
#62515=ORIENTED_EDGE ( 'NONE', *, *, #19166, .F. ) ;
#62516=VERTEX_POINT ( 'NONE', #54439 ) ;
#62518=VERTEX_POINT ( 'NONE', #115946 ) ;
#62519=ORIENTED_EDGE ( 'NONE', *, *, #99724, .T. ) ;
#62521=EDGE_LOOP ( 'NONE', ( #47132, #114901, #102234, #86280 ) ) ;
#62522=EDGE_LOOP ( 'NONE', ( #1631, #128890 ) ) ;
#62523=CIRCLE ( 'NONE', #6051, 0.1000000000000000056 ) ;
#62525=CARTESIAN_POINT ( 'NONE',  ( 14.66596006039096522, -2.499999999999999556, 7.515560524215777249 ) ) ;
#62526=DIRECTION ( 'NONE',  ( -0.000000000000000000, 1.000000000000000000, -0.000000000000000000 ) ) ;
#62527=CARTESIAN_POINT ( 'NONE',  ( -12.89999999999999147, 2.500000000000000000, -4.230127018922199333 ) ) ;
#62528=CIRCLE ( 'NONE', #79241, 0.06509327318403745899 ) ;
#62529=VERTEX_POINT ( 'NONE', #105491 ) ;
#62530=DIRECTION ( 'NONE',  ( 0.000000000000000000, 0.000000000000000000, -1.000000000000000000 ) ) ;
#62531=ORIENTED_EDGE ( 'NONE', *, *, #82969, .T. ) ;
#62532=ORIENTED_EDGE ( 'NONE', *, *, #87247, .F. ) ;
#62533=VECTOR ( 'NONE', #21329, 1000.000000000000000 ) ;
#62534=DIRECTION ( 'NONE',  ( 0.000000000000000000, -0.000000000000000000, 1.000000000000000000 ) ) ;
#62535=CARTESIAN_POINT ( 'NONE',  ( -6.249999999999984901, 2.500000000000000000, -6.495190528383302464 ) ) ;
#62536=ORIENTED_EDGE ( 'NONE', *, *, #123113, .F. ) ;
#62537=VECTOR ( 'NONE', #95858, 1000.000000000000000 ) ;
#62538=ORIENTED_EDGE ( 'NONE', *, *, #66993, .F. ) ;
#62539=DIRECTION ( 'NONE',  ( -0.000000000000000000, -1.000000000000000000, -0.000000000000000000 ) ) ;
#62541=DIRECTION ( 'NONE',  ( -4.274815082592931898E-19, -0.9999939076577903929, -0.003490651415223739937 ) ) ;
#62542=CARTESIAN_POINT ( 'NONE',  ( 8.349999999999923261, 2.500000000000000000, -6.595190528383302109 ) ) ;
#62543=LINE ( 'NONE', #40979, #79624 ) ;
#62544=DIRECTION ( 'NONE',  ( -0.000000000000000000, 1.000000000000000000, -0.000000000000000000 ) ) ;
#62545=AXIS2_PLACEMENT_3D ( 'NONE', #83453, #123361, #15319 ) ;
#62546=VERTEX_POINT ( 'NONE', #16428 ) ;
#62547=CARTESIAN_POINT ( 'NONE',  ( 15.40585131959743848, -2.500000000000000000, 5.817868759122586830 ) ) ;
#62548=ADVANCED_FACE ( 'NONE', ( #55735 ), #126912, .T. ) ;
#62549=ORIENTED_EDGE ( 'NONE', *, *, #41212, .T. ) ;
#62550=CARTESIAN_POINT ( 'NONE',  ( 17.50000000000000000, 2.499999999999999556, -1.333333333333329929 ) ) ;
#62551=VECTOR ( 'NONE', #18453, 1000.000000000000000 ) ;
#62552=AXIS2_PLACEMENT_3D ( 'NONE', #108487, #117002, #47650 ) ;
#62553=DIRECTION ( 'NONE',  ( 0.000000000000000000, 0.000000000000000000, -1.000000000000000000 ) ) ;
#62554=DIRECTION ( 'NONE',  ( 0.000000000000000000, 0.000000000000000000, 1.000000000000000000 ) ) ;
#62555=FACE_OUTER_BOUND ( 'NONE', #116515, .T. ) ;
#62556=EDGE_CURVE ( 'NONE', #98451, #4284, #97657, .T. ) ;
#62557=CARTESIAN_POINT ( 'NONE',  ( -13.74999999999995381, 2.500000000000000000, 2.265063509461101354 ) ) ;
#62558=ADVANCED_FACE ( 'NONE', ( #124486 ), #41245, .T. ) ;
#62559=ORIENTED_EDGE ( 'NONE', *, *, #124463, .F. ) ;
#62560=DIRECTION ( 'NONE',  ( 0.000000000000000000, 0.000000000000000000, -1.000000000000000000 ) ) ;
#62561=AXIS2_PLACEMENT_3D ( 'NONE', #75736, #123544, #115659 ) ;
#62562=VECTOR ( 'NONE', #94617, 1000.000000000000000 ) ;
#62563=ADVANCED_FACE ( 'NONE', ( #26288 ), #49556, .T. ) ;
#62564=PLANE ( 'NONE',  #111469 ) ;
#62565=VERTEX_POINT ( 'NONE', #44632 ) ;
#62566=ADVANCED_FACE ( 'NONE', ( #34178 ), #83011, .T. ) ;
#62567=EDGE_LOOP ( 'NONE', ( #41, #65889 ) ) ;
#62569=CARTESIAN_POINT ( 'NONE',  ( 17.50000000000000000, -2.750000000000000444, 4.000000000000001776 ) ) ;
#62570=CARTESIAN_POINT ( 'NONE',  ( -4.999999999999986677, 2.500000000000000000, -0.1000000000000022815 ) ) ;
#62573=CARTESIAN_POINT ( 'NONE',  ( 5.399999999999936406, 12.50000000000000000, -3.702399969078687292 ) ) ;
#62574=CARTESIAN_POINT ( 'NONE',  ( -14.59999999999998366, 12.50000000000000000, -0.6928203230275520319 ) ) ;
#62575=DIRECTION ( 'NONE',  ( 0.000000000000000000, 1.000000000000000000, 0.000000000000000000 ) ) ;
#62576=DIRECTION ( 'NONE',  ( -0.000000000000000000, 1.000000000000000000, -0.000000000000000000 ) ) ;
#62577=CIRCLE ( 'NONE', #125252, 0.06509327318403745899 ) ;
#62578=CARTESIAN_POINT ( 'NONE',  ( -4.150000000000025224, 12.50000000000000000, 2.792790559304612064 ) ) ;
#62579=VECTOR ( 'NONE', #43763, 1000.000000000000000 ) ;
#62580=ORIENTED_EDGE ( 'NONE', *, *, #57078, .T. ) ;
#62581=CARTESIAN_POINT ( 'NONE',  ( -1.250000000000001110, 2.500000000000000000, -6.395190528383301931 ) ) ;
#62582=FACE_OUTER_BOUND ( 'NONE', #49274, .T. ) ;
#62583=DIRECTION ( 'NONE',  ( -0.000000000000000000, 1.000000000000000000, -0.000000000000000000 ) ) ;
#62584=DIRECTION ( 'NONE',  ( 0.000000000000000000, 0.000000000000000000, -1.000000000000000000 ) ) ;
#62585=AXIS2_PLACEMENT_3D ( 'NONE', #87182, #116006, #97658 ) ;
#62586=ORIENTED_EDGE ( 'NONE', *, *, #21229, .F. ) ;
#62587=AXIS2_PLACEMENT_3D ( 'NONE', #17440, #57390, #8273 ) ;
#62588=DIRECTION ( 'NONE',  ( 0.000000000000000000, 0.000000000000000000, 1.000000000000000000 ) ) ;
#62589=AXIS2_PLACEMENT_3D ( 'NONE', #99555, #50437, #68135 ) ;
#62590=LINE ( 'NONE', #52748, #34598 ) ;
#62591=CARTESIAN_POINT ( 'NONE',  ( 7.899999999999924860, 2.500000000000000000, 3.737306695894644371 ) ) ;
#62592=ORIENTED_EDGE ( 'NONE', *, *, #120970, .T. ) ;
#62593=VECTOR ( 'NONE', #15256, 1000.000000000000000 ) ;
#62594=ORIENTED_EDGE ( 'NONE', *, *, #66063, .T. ) ;
#62596=AXIS2_PLACEMENT_3D ( 'NONE', #101047, #81420, #11374 ) ;
#62597=VECTOR ( 'NONE', #59730, 1000.000000000000000 ) ;
#62598=ORIENTED_EDGE ( 'NONE', *, *, #14658, .F. ) ;
#62599=ORIENTED_EDGE ( 'NONE', *, *, #103718, .F. ) ;
#62600=CARTESIAN_POINT ( 'NONE',  ( -3.550000000000027800, 2.500000000000000000, 6.048780366869520364 ) ) ;
#62601=ADVANCED_FACE ( 'NONE', ( #19685 ), #18230, .T. ) ;
#62602=EDGE_CURVE ( 'NONE', #79916, #92862, #29505, .T. ) ;
#62603=CARTESIAN_POINT ( 'NONE',  ( 18.09676523922475511, 2.526776815559031331, -2.684906793686053561 ) ) ;
#62604=PLANE ( 'NONE',  #40062 ) ;
#62606=CARTESIAN_POINT ( 'NONE',  ( 8.749999999999921840, 12.50000000000000000, -5.802370205355749988 ) ) ;
#62607=ORIENTED_EDGE ( 'NONE', *, *, #53003, .F. ) ;
#62608=DIRECTION ( 'NONE',  ( 0.000000000000000000, 1.000000000000000000, 0.000000000000000000 ) ) ;
#62609=FACE_OUTER_BOUND ( 'NONE', #96871, .T. ) ;
#62610=ORIENTED_EDGE ( 'NONE', *, *, #35531, .T. ) ;
#62611=VECTOR ( 'NONE', #117367, 1000.000000000000000 ) ;
#62612=ADVANCED_FACE ( 'NONE', ( #88400 ), #22371, .T. ) ;
#62614=ADVANCED_FACE ( 'NONE', ( #116579 ), #48496, .T. ) ;
#62615=CARTESIAN_POINT ( 'NONE',  ( 7.099999999999927702, 12.50000000000000000, 5.022947341949748790 ) ) ;
#62616=EDGE_CURVE ( 'NONE', #29998, #34079, #124855, .T. ) ;
#62617=EDGE_LOOP ( 'NONE', ( #14757, #92189 ) ) ;
#62618=EDGE_CURVE ( 'NONE', #59390, #18883, #116424, .T. ) ;
#62619=ADVANCED_FACE ( 'NONE', ( #107413 ), #118485, .T. ) ;
#62620=EDGE_LOOP ( 'NONE', ( #61432, #874 ) ) ;
#62621=ORIENTED_EDGE ( 'NONE', *, *, #59204, .F. ) ;
#62622=ORIENTED_EDGE ( 'NONE', *, *, #46082, .T. ) ;
#62623=DIRECTION ( 'NONE',  ( -4.274815082592931898E-19, -0.9999939076577903929, -0.003490651415223739937 ) ) ;
#62624=CARTESIAN_POINT ( 'NONE',  ( 12.31005523291756809, 2.499999999999999556, 7.488833080794197627 ) ) ;
#62625=DIRECTION ( 'NONE',  ( 0.000000000000000000, 1.000000000000000000, 0.000000000000000000 ) ) ;
#62626=FACE_BOUND ( 'NONE', #70173, .T. ) ;
#62627=ORIENTED_EDGE ( 'NONE', *, *, #12907, .F. ) ;
#62629=AXIS2_PLACEMENT_3D ( 'NONE', #72209, #112130, #22475 ) ;
#62630=ADVANCED_FACE ( 'NONE', ( #127695 ), #76735, .T. ) ;
#62631=CARTESIAN_POINT ( 'NONE',  ( -8.150000000000009237, 2.500000000000000000, 6.148780366869520009 ) ) ;
#62632=DIRECTION ( 'NONE',  ( 0.000000000000000000, 0.000000000000000000, -1.000000000000000000 ) ) ;
#62633=DIRECTION ( 'NONE',  ( 0.000000000000000000, 0.000000000000000000, -1.000000000000000000 ) ) ;
#62634=DIRECTION ( 'NONE',  ( 0.6795087154617358571, 9.398010995470537367E-14, -0.7336674352944538846 ) ) ;
#62635=AXIS2_PLACEMENT_3D ( 'NONE', #41450, #80719, #90517 ) ;
#62636=CARTESIAN_POINT ( 'NONE',  ( -3.150000000000030109, 12.50000000000000000, -2.511473670974877948 ) ) ;
#62637=CARTESIAN_POINT ( 'NONE',  ( -1.850000000000033840, 2.500000000000000000, 6.248780366869521430 ) ) ;
#62638=CIRCLE ( 'NONE', #114841, 0.06509327318403745899 ) ;
#62639=AXIS2_PLACEMENT_3D ( 'NONE', #104466, #122829, #32535 ) ;
#62640=EDGE_LOOP ( 'NONE', ( #105420, #10824, #26706, #3687 ) ) ;
#62641=ORIENTED_EDGE ( 'NONE', *, *, #124497, .F. ) ;
#62642=ORIENTED_EDGE ( 'NONE', *, *, #101142, .F. ) ;
#62643=ORIENTED_EDGE ( 'NONE', *, *, #102989, .T. ) ;
#62644=ORIENTED_EDGE ( 'NONE', *, *, #5764, .T. ) ;
#62645=LINE ( 'NONE', #3702, #14618 ) ;
#62646=CIRCLE ( 'NONE', #29205, 0.1000000000000000472 ) ;
#62647=DIRECTION ( 'NONE',  ( 0.000000000000000000, -0.000000000000000000, 1.000000000000000000 ) ) ;
#62648=VERTEX_POINT ( 'NONE', #71339 ) ;
#62649=FACE_BOUND ( 'NONE', #84097, .T. ) ;
#62650=CARTESIAN_POINT ( 'NONE',  ( -1.650000000000034772, 12.50000000000000000, 6.495190528383297135 ) ) ;
#62652=AXIS2_PLACEMENT_3D ( 'NONE', #76926, #87373, #85446 ) ;
#62653=ORIENTED_EDGE ( 'NONE', *, *, #71914, .T. ) ;
#62654=DIRECTION ( 'NONE',  ( 0.000000000000000000, -0.9999939076577903929, 0.003490651415223739937 ) ) ;
#62655=DIRECTION ( 'NONE',  ( 0.000000000000000000, -0.000000000000000000, 1.000000000000000000 ) ) ;
#62656=LINE ( 'NONE', #94035, #60037 ) ;
#62657=ORIENTED_EDGE ( 'NONE', *, *, #3650, .F. ) ;
#62659=EDGE_LOOP ( 'NONE', ( #63729, #102337, #127911, #115813 ) ) ;
#62660=EDGE_CURVE ( 'NONE', #34783, #115836, #90998, .T. ) ;
#62661=ORIENTED_EDGE ( 'NONE', *, *, #83241, .T. ) ;
#62662=ORIENTED_EDGE ( 'NONE', *, *, #22671, .F. ) ;
#62663=CIRCLE ( 'NONE', #108615, 0.06509327318403745899 ) ;
#62664=CARTESIAN_POINT ( 'NONE',  ( -6.249999999999984901, 12.50000000000000000, -2.230156782645139391 ) ) ;
#62665=FACE_OUTER_BOUND ( 'NONE', #88289, .T. ) ;
#62666=CARTESIAN_POINT ( 'NONE',  ( -0.4000000000000396572, 2.500000000000000000, 3.637306695894644726 ) ) ;
#62667=ORIENTED_EDGE ( 'NONE', *, *, #125933, .T. ) ;
#62668=DIRECTION ( 'NONE',  ( 0.000000000000000000, 0.000000000000000000, 1.000000000000000000 ) ) ;
#62669=AXIS2_PLACEMENT_3D ( 'NONE', #31462, #110652, #22301 ) ;
#62671=AXIS2_PLACEMENT_3D ( 'NONE', #94747, #73183, #64007 ) ;
#62672=DIRECTION ( 'NONE',  ( 0.000000000000000000, 0.000000000000000000, 1.000000000000000000 ) ) ;
#62673=DIRECTION ( 'NONE',  ( 0.000000000000000000, 1.000000000000000000, 0.000000000000000000 ) ) ;
#62674=ORIENTED_EDGE ( 'NONE', *, *, #106007, .T. ) ;
#62675=ADVANCED_FACE ( 'NONE', ( #2595 ), #20966, .T. ) ;
#62676=DIRECTION ( 'NONE',  ( 0.000000000000000000, 1.000000000000000000, 0.000000000000000000 ) ) ;
#62677=VECTOR ( 'NONE', #738, 1000.000000000000000 ) ;
#62678=EDGE_LOOP ( 'NONE', ( #19848, #88616 ) ) ;
#62679=CARTESIAN_POINT ( 'NONE',  ( 3.099999999999945022, 12.50000000000000000, -0.3464101615137783474 ) ) ;
#62680=CIRCLE ( 'NONE', #28946, 0.1000000000000002554 ) ;
#62681=AXIS2_PLACEMENT_3D ( 'NONE', #60909, #49186, #128390 ) ;
#62682=ORIENTED_EDGE ( 'NONE', *, *, #46942, .F. ) ;
#62683=ORIENTED_EDGE ( 'NONE', *, *, #106217, .T. ) ;
#62684=DIRECTION ( 'NONE',  ( 0.000000000000000000, 0.000000000000000000, -1.000000000000000000 ) ) ;
#62685=FACE_OUTER_BOUND ( 'NONE', #873, .T. ) ;
#62686=PLANE ( 'NONE',  #6950 ) ;
#62687=CARTESIAN_POINT ( 'NONE',  ( 13.29999999999990301, 2.500000000000000000, -4.430127018922202176 ) ) ;
#62688=DIRECTION ( 'NONE',  ( -0.000000000000000000, 1.000000000000000000, -0.000000000000000000 ) ) ;
#62689=EDGE_LOOP ( 'NONE', ( #125515, #53240 ) ) ;
#62690=ORIENTED_EDGE ( 'NONE', *, *, #67560, .F. ) ;
#62692=LINE ( 'NONE', #30663, #60233 ) ;
#62693=FACE_OUTER_BOUND ( 'NONE', #83694, .T. ) ;
#62694=CARTESIAN_POINT ( 'NONE',  ( 12.09999999999990195, 12.50000000000000000, 0.06509327318403515528 ) ) ;
#62695=VERTEX_POINT ( 'NONE', #111930 ) ;
#62696=EDGE_LOOP ( 'NONE', ( #73543, #106048 ) ) ;
#62697=FACE_OUTER_BOUND ( 'NONE', #59139, .T. ) ;
#62698=CONICAL_SURFACE ( 'NONE', #8293, 0.1000000000000000472, 0.003490658503988666988 ) ;
#62699=EDGE_LOOP ( 'NONE', ( #15462, #7060, #85072, #56272 ) ) ;
#62700=DIRECTION ( 'NONE',  ( 0.000000000000000000, 0.000000000000000000, 1.000000000000000000 ) ) ;
#62701=DIRECTION ( 'NONE',  ( -0.000000000000000000, -1.000000000000000000, -0.000000000000000000 ) ) ;
#62702=EDGE_CURVE ( 'NONE', #19796, #103770, #21616, .T. ) ;
#62703=DIRECTION ( 'NONE',  ( 0.000000000000000000, 0.000000000000000000, 1.000000000000000000 ) ) ;
#62704=ORIENTED_EDGE ( 'NONE', *, *, #68480, .F. ) ;
#62705=PLANE ( 'NONE',  #39877 ) ;
#62706=CARTESIAN_POINT ( 'NONE',  ( 5.849999999999931255, 2.500000000000000000, 2.857883832488649301 ) ) ;
#62707=CARTESIAN_POINT ( 'NONE',  ( -12.49999999999999289, 2.500000000000000000, 3.637306695894644726 ) ) ;
#62708=AXIS2_PLACEMENT_3D ( 'NONE', #4003, #5288, #34132 ) ;
#62709=CARTESIAN_POINT ( 'NONE',  ( 11.89999999999990443, 12.50000000000000000, 0.3464101615137736845 ) ) ;
#62710=PLANE ( 'NONE',  #64624 ) ;
#62711=ADVANCED_FACE ( 'NONE', ( #51728 ), #675, .T. ) ;
#62712=ORIENTED_EDGE ( 'NONE', *, *, #24349, .T. ) ;
#62713=CARTESIAN_POINT ( 'NONE',  ( -14.14999999999998614, 2.500000000000000000, -2.857883832488651521 ) ) ;
#62714=CARTESIAN_POINT ( 'NONE',  ( 87.50000000000001421, -3.974992050023846257, 6.359987280038162716 ) ) ;
#62715=EDGE_CURVE ( 'NONE', #6628, #107306, #90328, .T. ) ;
#62716=VERTEX_POINT ( 'NONE', #61550 ) ;
#62718=ORIENTED_EDGE ( 'NONE', *, *, #101038, .T. ) ;
#62719=ADVANCED_FACE ( 'NONE', ( #81808 ), #122792, .T. ) ;
#62721=CARTESIAN_POINT ( 'NONE',  ( -10.40000000000000213, 2.500000000000000000, 5.122947341949749323 ) ) ;
#62722=EDGE_CURVE ( 'NONE', #37252, #123620, #91639, .T. ) ;
#62723=ADVANCED_FACE ( 'NONE', ( #111252 ), #35073, .T. ) ;
#62725=CARTESIAN_POINT ( 'NONE',  ( -7.950000000000012612, 2.500000000000000000, 2.265063509461097357 ) ) ;
#62726=DIRECTION ( 'NONE',  ( 0.000000000000000000, 1.000000000000000000, 0.000000000000000000 ) ) ;
#62727=CARTESIAN_POINT ( 'NONE',  ( 7.299999999999926104, 2.500000000000000000, -0.3464101615137782364 ) ) ;
#62728=DIRECTION ( 'NONE',  ( 0.000000000000000000, 0.000000000000000000, 1.000000000000000000 ) ) ;
#62729=CARTESIAN_POINT ( 'NONE',  ( 12.89999999999989910, 2.500000000000000000, -0.5928203230275542746 ) ) ;
#62730=AXIS2_PLACEMENT_3D ( 'NONE', #85687, #37256, #56856 ) ;
#62731=EDGE_CURVE ( 'NONE', #39246, #5618, #116522, .T. ) ;
#62732=PLANE ( 'NONE',  #70973 ) ;
#62733=VERTEX_POINT ( 'NONE', #102110 ) ;
#62734=EDGE_CURVE ( 'NONE', #80247, #14617, #30160, .T. ) ;
#62735=ORIENTED_EDGE ( 'NONE', *, *, #21225, .F. ) ;
#62736=AXIS2_PLACEMENT_3D ( 'NONE', #63212, #13460, #93325 ) ;
#62737=AXIS2_PLACEMENT_3D ( 'NONE', #4308, #93367, #123455 ) ;
#62738=ORIENTED_EDGE ( 'NONE', *, *, #13295, .T. ) ;
#62739=EDGE_LOOP ( 'NONE', ( #29310, #65185 ) ) ;
#62740=CARTESIAN_POINT ( 'NONE',  ( 10.64999999999991331, 12.50000000000000000, -2.511473670974877948 ) ) ;
#62741=DIRECTION ( 'NONE',  ( 0.000000000000000000, 1.000000000000000000, 0.000000000000000000 ) ) ;
#62742=AXIS2_PLACEMENT_3D ( 'NONE', #91866, #44051, #114714 ) ;
#62743=CIRCLE ( 'NONE', #14591, 0.1000000000000002554 ) ;
#62744=ORIENTED_EDGE ( 'NONE', *, *, #104778, .F. ) ;
#62746=CARTESIAN_POINT ( 'NONE',  ( -7.100000000000013856, 2.500000000000000000, 3.637306695894644726 ) ) ;
#62747=CARTESIAN_POINT ( 'NONE',  ( -8.950000000000008171, 12.50000000000000000, 1.883746621131358934 ) ) ;
#62748=ORIENTED_EDGE ( 'NONE', *, *, #36312, .T. ) ;
#62749=CARTESIAN_POINT ( 'NONE',  ( -12.09999999999999609, 2.500000000000000000, -4.430127018922199511 ) ) ;
#62750=DIRECTION ( 'NONE',  ( 0.000000000000000000, 1.000000000000000000, 0.000000000000000000 ) ) ;
#62751=ORIENTED_EDGE ( 'NONE', *, *, #41884, .T. ) ;
#62752=ORIENTED_EDGE ( 'NONE', *, *, #93173, .T. ) ;
#62753=ORIENTED_EDGE ( 'NONE', *, *, #115140, .F. ) ;
#62754=VERTEX_POINT ( 'NONE', #11784 ) ;
#62755=DIRECTION ( 'NONE',  ( 0.000000000000000000, 0.000000000000000000, 1.000000000000000000 ) ) ;
#62756=DIRECTION ( 'NONE',  ( 0.000000000000000000, 0.000000000000000000, -1.000000000000000000 ) ) ;
#62757=DIRECTION ( 'NONE',  ( 0.000000000000000000, 0.000000000000000000, 1.000000000000000000 ) ) ;
#62758=ADVANCED_FACE ( 'NONE', ( #32096 ), #64298, .T. ) ;
#62759=DIRECTION ( 'NONE',  ( -0.000000000000000000, -1.000000000000000000, -0.000000000000000000 ) ) ;
#62760=CONICAL_SURFACE ( 'NONE', #25090, 0.1000000000000002554, 0.003490658503988666988 ) ;
#62761=VERTEX_POINT ( 'NONE', #82481 ) ;
#62762=EDGE_CURVE ( 'NONE', #110935, #22979, #118672, .T. ) ;
#62763=FACE_OUTER_BOUND ( 'NONE', #88473, .T. ) ;
#62764=ORIENTED_EDGE ( 'NONE', *, *, #112579, .T. ) ;
#62765=FACE_OUTER_BOUND ( 'NONE', #88947, .T. ) ;
#62766=LINE ( 'NONE', #52295, #104026 ) ;
#62767=CARTESIAN_POINT ( 'NONE',  ( 6.849999999999930367, 2.500000000000000000, -6.048780366869526581 ) ) ;
#62768=FACE_OUTER_BOUND ( 'NONE', #109022, .T. ) ;
#62769=EDGE_CURVE ( 'NONE', #129537, #76489, #29929, .T. ) ;
#62770=CONICAL_SURFACE ( 'NONE', #64806, 0.1000000000000002554, 0.003490658503988666988 ) ;
#62771=EDGE_CURVE ( 'NONE', #33584, #89626, #50218, .T. ) ;
#62772=EDGE_LOOP ( 'NONE', ( #38554, #9436 ) ) ;
#62773=ADVANCED_FACE ( 'NONE', ( #69847 ), #70556, .T. ) ;
#62774=ORIENTED_EDGE ( 'NONE', *, *, #103669, .F. ) ;
#62775=ORIENTED_EDGE ( 'NONE', *, *, #125876, .F. ) ;
#62776=CARTESIAN_POINT ( 'NONE',  ( 6.049999999999930544, 12.50000000000000000, 2.576566944158910744 ) ) ;
#62777=DIRECTION ( 'NONE',  ( 0.000000000000000000, 0.000000000000000000, 1.000000000000000000 ) ) ;
#62778=CARTESIAN_POINT ( 'NONE',  ( 4.599999999999936584, 12.50000000000000000, 3.572213422710607489 ) ) ;
#62779=FACE_BOUND ( 'NONE', #94245, .T. ) ;
#62780=AXIS2_PLACEMENT_3D ( 'NONE', #26250, #40436, #126379 ) ;
#62781=CARTESIAN_POINT ( 'NONE',  ( -6.250000000000021316, 12.50000000000000000, -5.802370205355749988 ) ) ;
#62782=DIRECTION ( 'NONE',  ( -0.000000000000000000, 1.000000000000000000, -0.000000000000000000 ) ) ;
#62783=EDGE_CURVE ( 'NONE', #89626, #6313, #28808, .T. ) ;
#62784=CARTESIAN_POINT ( 'NONE',  ( 2.299999999999948752, 12.50000000000000000, 0.4115034346978109769 ) ) ;
#62785=CIRCLE ( 'NONE', #23063, 0.06509327318403743123 ) ;
#62786=AXIS2_PLACEMENT_3D ( 'NONE', #37813, #48936, #77718 ) ;
#62789=DIRECTION ( 'NONE',  ( 0.000000000000000000, 0.000000000000000000, 1.000000000000000000 ) ) ;
#62790=ORIENTED_EDGE ( 'NONE', *, *, #11742, .F. ) ;
#62791=CIRCLE ( 'NONE', #37742, 0.1000000000000002554 ) ;
#62792=LINE ( 'NONE', #15596, #99519 ) ;
#62793=CIRCLE ( 'NONE', #16691, 0.06509327318403745899 ) ;
#62794=EDGE_LOOP ( 'NONE', ( #61950, #81273, #111343, #116406 ) ) ;
#62795=ORIENTED_EDGE ( 'NONE', *, *, #99190, .T. ) ;
#62796=CARTESIAN_POINT ( 'NONE',  ( 14.59999999999989484, 2.500000000000000000, -2.276824562219559311E-15 ) ) ;
#62797=CARTESIAN_POINT ( 'NONE',  ( -7.500000000000016875, 2.500000000000000000, 0.7928203230275495672 ) ) ;
#62798=EDGE_CURVE ( 'NONE', #23803, #27914, #129440, .T. ) ;
#62799=FACE_BOUND ( 'NONE', #38044, .T. ) ;
#62800=DIRECTION ( 'NONE',  ( -0.000000000000000000, 1.000000000000000000, -0.000000000000000000 ) ) ;
#62801=VERTEX_POINT ( 'NONE', #39127 ) ;
#62802=CARTESIAN_POINT ( 'NONE',  ( -12.29999999999999716, 12.50000000000000000, -3.983716857408423628 ) ) ;
#62803=LINE ( 'NONE', #102702, #22779 ) ;
#62804=ORIENTED_EDGE ( 'NONE', *, *, #31382, .F. ) ;
#62805=DIRECTION ( 'NONE',  ( -0.000000000000000000, -1.000000000000000000, -0.000000000000000000 ) ) ;
#62806=CARTESIAN_POINT ( 'NONE',  ( 5.399999999999932854, 12.50000000000000000, 5.022947341949748790 ) ) ;
#62807=ADVANCED_FACE ( 'NONE', ( #48270 ), #114469, .T. ) ;
#62808=CIRCLE ( 'NONE', #29369, 0.06509327318403745899 ) ;
#62809=ORIENTED_EDGE ( 'NONE', *, *, #19225, .T. ) ;
#62810=DIRECTION ( 'NONE',  ( 0.000000000000000000, 0.000000000000000000, 1.000000000000000000 ) ) ;
#62811=AXIS2_PLACEMENT_3D ( 'NONE', #36466, #106466, #16130 ) ;
#62812=DIRECTION ( 'NONE',  ( 0.000000000000000000, 0.000000000000000000, 1.000000000000000000 ) ) ;
#62813=EDGE_LOOP ( 'NONE', ( #13846, #106562, #17092, #61119 ) ) ;
#62814=DIRECTION ( 'NONE',  ( 0.000000000000000000, 1.000000000000000000, 0.000000000000000000 ) ) ;
#62815=VECTOR ( 'NONE', #32978, 1000.000000000000000 ) ;
#62816=CONICAL_SURFACE ( 'NONE', #117079, 0.1000000000000002554, 0.003490658503988666988 ) ;
#62818=CARTESIAN_POINT ( 'NONE',  ( 8.749999999999923617, 12.50000000000000000, -7.188010851410854052 ) ) ;
#62819=ORIENTED_EDGE ( 'NONE', *, *, #72373, .F. ) ;
#62820=ORIENTED_EDGE ( 'NONE', *, *, #33174, .F. ) ;
#62821=EDGE_CURVE ( 'NONE', #17776, #16630, #18156, .T. ) ;
#62823=ORIENTED_EDGE ( 'NONE', *, *, #72157, .F. ) ;
#62824=CARTESIAN_POINT ( 'NONE',  ( -6.850000000000013856, 2.500000000000000000, 1.718653347947321386 ) ) ;
#62825=DIRECTION ( 'NONE',  ( -0.000000000000000000, -1.000000000000000000, -0.000000000000000000 ) ) ;
#62826=VERTEX_POINT ( 'NONE', #128127 ) ;
#62828=FACE_OUTER_BOUND ( 'NONE', #107974, .T. ) ;
#62829=DIRECTION ( 'NONE',  ( -0.000000000000000000, -1.000000000000000000, -0.000000000000000000 ) ) ;
#62832=EDGE_LOOP ( 'NONE', ( #99138, #90717, #68305, #36933 ) ) ;
#62833=ORIENTED_EDGE ( 'NONE', *, *, #92188, .F. ) ;
#62834=DIRECTION ( 'NONE',  ( -0.000000000000000000, 1.000000000000000000, -0.000000000000000000 ) ) ;
#62835=ORIENTED_EDGE ( 'NONE', *, *, #126328, .F. ) ;
#62836=CARTESIAN_POINT ( 'NONE',  ( -5.400000000000019895, 2.500000000000000000, -0.6928203230275541413 ) ) ;
#62837=ORIENTED_EDGE ( 'NONE', *, *, #109523, .T. ) ;
#62838=ORIENTED_EDGE ( 'NONE', *, *, #109411, .T. ) ;
#62839=VERTEX_POINT ( 'NONE', #87540 ) ;
#62840=CARTESIAN_POINT ( 'NONE',  ( 0.6499999999999561684, 12.50000000000000000, 2.511473670974873507 ) ) ;
#62841=AXIS2_PLACEMENT_3D ( 'NONE', #60326, #21673, #62248 ) ;
#62843=CONICAL_SURFACE ( 'NONE', #52378, 0.1000000000000000056, 0.003490658503988666988 ) ;
#62844=CARTESIAN_POINT ( 'NONE',  ( -14.99999999999998401, 12.50000000000000000, 0.6928203230275518099 ) ) ;
#62845=EDGE_CURVE ( 'NONE', #14124, #84685, #74774, .T. ) ;
#62846=CARTESIAN_POINT ( 'NONE',  ( -5.400000000000019895, 12.50000000000000000, 4.330127018922196314 ) ) ;
#62847=DIRECTION ( 'NONE',  ( 0.000000000000000000, 0.000000000000000000, -1.000000000000000000 ) ) ;
#62848=PLANE ( 'NONE',  #29780 ) ;
#62849=DIRECTION ( 'NONE',  ( 0.000000000000000000, 1.000000000000000000, 0.000000000000000000 ) ) ;
#62850=DIRECTION ( 'NONE',  ( 0.000000000000000000, 0.000000000000000000, 1.000000000000000000 ) ) ;
#62851=CARTESIAN_POINT ( 'NONE',  ( -4.150000000000024336, 12.50000000000000000, 2.099970236277060032 ) ) ;
#62852=AXIS2_PLACEMENT_3D ( 'NONE', #86892, #128786, #56138 ) ;
#62853=EDGE_CURVE ( 'NONE', #83526, #126341, #104015, .T. ) ;
#62854=ORIENTED_EDGE ( 'NONE', *, *, #31123, .F. ) ;
#62855=CARTESIAN_POINT ( 'NONE',  ( -16.50000000000000000, -2.500000000000000000, 1.734723475976807094E-15 ) ) ;
#62856=ADVANCED_FACE ( 'NONE', ( #20103 ), #118578, .T. ) ;
#62857=ORIENTED_EDGE ( 'NONE', *, *, #102191, .T. ) ;
#62858=EDGE_CURVE ( 'NONE', #87021, #101722, #60122, .T. ) ;
#62859=ORIENTED_EDGE ( 'NONE', *, *, #21775, .F. ) ;
#62860=EDGE_CURVE ( 'NONE', #50743, #34595, #8976, .T. ) ;
#62861=DIRECTION ( 'NONE',  ( 0.000000000000000000, 0.000000000000000000, -1.000000000000000000 ) ) ;
#62862=DIRECTION ( 'NONE',  ( 0.000000000000000000, 0.000000000000000000, 1.000000000000000000 ) ) ;
#62863=EDGE_CURVE ( 'NONE', #121543, #55871, #95604, .T. ) ;
#62864=DIRECTION ( 'NONE',  ( 0.000000000000000000, 0.000000000000000000, -1.000000000000000000 ) ) ;
#62865=AXIS2_PLACEMENT_3D ( 'NONE', #29430, #99465, #9777 ) ;
#62866=CARTESIAN_POINT ( 'NONE',  ( 1.249999999999952038, 2.500000000000000000, -1.372243186433550033 ) ) ;
#62867=VECTOR ( 'NONE', #110414, 1000.000000000000000 ) ;
#62868=DIRECTION ( 'NONE',  ( 0.000000000000000000, 1.000000000000000000, 0.000000000000000000 ) ) ;
#62869=ADVANCED_FACE ( 'NONE', ( #19445 ), #39198, .T. ) ;
#62870=DIRECTION ( 'NONE',  ( 0.000000000000000000, 1.000000000000000000, 0.000000000000000000 ) ) ;
#62871=EDGE_CURVE ( 'NONE', #16061, #40173, #53843, .T. ) ;
#62872=DIRECTION ( 'NONE',  ( -0.000000000000000000, -1.000000000000000000, -0.000000000000000000 ) ) ;
#62873=EDGE_LOOP ( 'NONE', ( #285, #74770, #109958, #60690 ) ) ;
#62874=ADVANCED_FACE ( 'NONE', ( #27320 ), #7854, .T. ) ;
#62875=EDGE_CURVE ( 'NONE', #116833, #49326, #58057, .T. ) ;
#62876=CIRCLE ( 'NONE', #52402, 0.09999999999999982514 ) ;
#62877=EDGE_CURVE ( 'NONE', #80574, #84780, #55885, .T. ) ;
#62878=ORIENTED_EDGE ( 'NONE', *, *, #88422, .F. ) ;
#62879=ADVANCED_FACE ( 'NONE', ( #39765 ), #18321, .T. ) ;
#62880=ORIENTED_EDGE ( 'NONE', *, *, #74984, .F. ) ;
#62881=AXIS2_PLACEMENT_3D ( 'NONE', #97235, #7552, #9506 ) ;
#62882=ORIENTED_EDGE ( 'NONE', *, *, #83562, .T. ) ;
#62883=VERTEX_POINT ( 'NONE', #59658 ) ;
#62884=EDGE_CURVE ( 'NONE', #59076, #99205, #58983, .T. ) ;
#62885=FACE_OUTER_BOUND ( 'NONE', #108575, .T. ) ;
#62886=DIRECTION ( 'NONE',  ( 0.000000000000000000, 0.000000000000000000, -1.000000000000000000 ) ) ;
#62887=DIRECTION ( 'NONE',  ( 0.000000000000000000, 1.000000000000000000, 0.000000000000000000 ) ) ;
#62888=DIRECTION ( 'NONE',  ( -0.000000000000000000, -1.000000000000000000, -0.000000000000000000 ) ) ;
#62889=CARTESIAN_POINT ( 'NONE',  ( 3.349999999999941025, 12.50000000000000000, 7.188010851410848723 ) ) ;
#62890=EDGE_LOOP ( 'NONE', ( #62820, #68531 ) ) ;
#62891=CARTESIAN_POINT ( 'NONE',  ( -7.050000000000016698, 2.500000000000000000, -6.595190528383302109 ) ) ;
#62892=CARTESIAN_POINT ( 'NONE',  ( -1.850000000000033840, 2.500000000000000000, 6.148780366869520897 ) ) ;
#62893=CARTESIAN_POINT ( 'NONE',  ( -10.85000000000000142, 12.50000000000000000, -7.188010851410850499 ) ) ;
#62894=CARTESIAN_POINT ( 'NONE',  ( 14.79999999999989413, 2.500000000000000000, -0.4464101615137782142 ) ) ;
#62895=EDGE_LOOP ( 'NONE', ( #9286, #122839, #106084, #106659 ) ) ;
#62896=EDGE_LOOP ( 'NONE', ( #115051, #83812 ) ) ;
#62898=AXIS2_PLACEMENT_3D ( 'NONE', #54328, #81838, #82517 ) ;
#62899=DIRECTION ( 'NONE',  ( -0.000000000000000000, 1.000000000000000000, -0.000000000000000000 ) ) ;
#62900=AXIS2_PLACEMENT_3D ( 'NONE', #50013, #30369, #89908 ) ;
#62901=CONICAL_SURFACE ( 'NONE', #16881, 0.1000000000000002554, 0.003490658503988666988 ) ;
#62902=DIRECTION ( 'NONE',  ( 0.000000000000000000, -0.9999939076577903929, 0.003490651415223739937 ) ) ;
#62903=CARTESIAN_POINT ( 'NONE',  ( -0.8000000000000381251, 2.500000000000000000, 4.230127018922196669 ) ) ;
#62904=CONICAL_SURFACE ( 'NONE', #4286, 0.1000000000000002554, 0.003490658503988666988 ) ;
#62905=CONICAL_SURFACE ( 'NONE', #94283, 0.1000000000000002554, 0.003490658503988666988 ) ;
#62906=VERTEX_POINT ( 'NONE', #47881 ) ;
#62907=CARTESIAN_POINT ( 'NONE',  ( -10.00000000000000355, 2.500000000000000000, 3.537306695894645081 ) ) ;
#62908=DIRECTION ( 'NONE',  ( -0.000000000000000000, -1.000000000000000000, -0.000000000000000000 ) ) ;
#62909=DIRECTION ( 'NONE',  ( 0.000000000000000000, 1.000000000000000000, 0.000000000000000000 ) ) ;
#62910=CARTESIAN_POINT ( 'NONE',  ( -2.950000000000029932, 12.50000000000000000, -2.099970236277064473 ) ) ;
#62911=EDGE_CURVE ( 'NONE', #25124, #121281, #129086, .T. ) ;
#62912=CARTESIAN_POINT ( 'NONE',  ( 6.649999999999928413, 2.500000000000000000, 2.957883832488649389 ) ) ;
#62913=ADVANCED_FACE ( 'NONE', ( #119828 ), #10505, .T. ) ;
#62914=VERTEX_POINT ( 'NONE', #39366 ) ;
#62915=ORIENTED_EDGE ( 'NONE', *, *, #13510, .T. ) ;
#62916=CARTESIAN_POINT ( 'NONE',  ( -12.49999999999995737, 2.500000000000000000, 4.430127018922196847 ) ) ;
#62917=FACE_OUTER_BOUND ( 'NONE', #6808, .T. ) ;
#62918=CARTESIAN_POINT ( 'NONE',  ( 6.899999999999928413, 2.500000000000000000, -3.983716857408426293 ) ) ;
#62919=ADVANCED_FACE ( 'NONE', ( #69428 ), #97831, .T. ) ;
#62920=DIRECTION ( 'NONE',  ( 0.000000000000000000, 0.000000000000000000, 1.000000000000000000 ) ) ;
#62921=VERTEX_POINT ( 'NONE', #7930 ) ;
#62922=EDGE_LOOP ( 'NONE', ( #107425, #48365, #57848, #11167 ) ) ;
#62923=CARTESIAN_POINT ( 'NONE',  ( 5.399999999999935518, 12.50000000000000000, -4.265033745738164406 ) ) ;
#62924=DIRECTION ( 'NONE',  ( -4.274815082592931898E-19, -0.9999939076577903929, -0.003490651415223739937 ) ) ;
#62925=DIRECTION ( 'NONE',  ( 0.000000000000000000, 0.000000000000000000, 1.000000000000000000 ) ) ;
#62926=CARTESIAN_POINT ( 'NONE',  ( -1.650000000000034328, 2.500000000000000000, -6.495190528383302464 ) ) ;
#62927=EDGE_LOOP ( 'NONE', ( #100487, #6436, #115974, #30213 ) ) ;
#62928=VECTOR ( 'NONE', #120367, 1000.000000000000000 ) ;
#62929=FACE_OUTER_BOUND ( 'NONE', #113028, .T. ) ;
#62930=CIRCLE ( 'NONE', #44151, 0.1000000000000002554 ) ;
#62931=CARTESIAN_POINT ( 'NONE',  ( -11.44999999999999751, 2.500000000000000000, 6.941600689897073018 ) ) ;
#62932=ORIENTED_EDGE ( 'NONE', *, *, #31433, .T. ) ;
#62933=CARTESIAN_POINT ( 'NONE',  ( 9.999999999999914735, 2.500000000000000000, 0.6928203230275494784 ) ) ;
#62934=ORIENTED_EDGE ( 'NONE', *, *, #81501, .F. ) ;
#62935=AXIS2_PLACEMENT_3D ( 'NONE', #11345, #214, #41475 ) ;
#62936=DIRECTION ( 'NONE',  ( 0.000000000000000000, 1.000000000000000000, 0.000000000000000000 ) ) ;
#62937=AXIS2_PLACEMENT_3D ( 'NONE', #108732, #10525, #90370 ) ;
#62938=ORIENTED_EDGE ( 'NONE', *, *, #77105, .T. ) ;
#62939=CARTESIAN_POINT ( 'NONE',  ( -11.25000000000000178, 2.500000000000000000, -1.572243186433546214 ) ) ;
#62940=DIRECTION ( 'NONE',  ( 0.000000000000000000, -0.9999939076577903929, 0.003490651415223739937 ) ) ;
#62941=ORIENTED_EDGE ( 'NONE', *, *, #112935, .T. ) ;
#62942=ORIENTED_EDGE ( 'NONE', *, *, #7695, .F. ) ;
#62944=CARTESIAN_POINT ( 'NONE',  ( 14.39999999999989555, 2.500000000000000000, -0.2464101615137782308 ) ) ;
#62945=AXIS2_PLACEMENT_3D ( 'NONE', #26048, #5100, #16199 ) ;
#62948=AXIS2_PLACEMENT_3D ( 'NONE', #33788, #126021, #54078 ) ;
#62949=DIRECTION ( 'NONE',  ( -0.000000000000000000, 1.000000000000000000, -0.000000000000000000 ) ) ;
#62950=CARTESIAN_POINT ( 'NONE',  ( -12.09999999999999609, 2.500000000000000000, 0.6928203230275535862 ) ) ;
#62951=CARTESIAN_POINT ( 'NONE',  ( -1.900000000000034994, 2.500000000000000000, -4.676537180435978769 ) ) ;
#62952=CARTESIAN_POINT ( 'NONE',  ( -1.450000000000036371, 12.50000000000000000, 2.511473670974873507 ) ) ;
#62953=CARTESIAN_POINT ( 'NONE',  ( -9.350000000000008527, 2.500000000000000000, -6.841600689897072485 ) ) ;
#62954=AXIS2_PLACEMENT_3D ( 'NONE', #33168, #12834, #110416 ) ;
#62955=VERTEX_POINT ( 'NONE', #79276 ) ;
#62956=EDGE_LOOP ( 'NONE', ( #27148, #82585 ) ) ;
#62957=DIRECTION ( 'NONE',  ( 0.000000000000000000, -0.9999939076577903929, 0.003490651415223739937 ) ) ;
#62958=EDGE_LOOP ( 'NONE', ( #9088, #104268, #85998, #25017 ) ) ;
#62959=CIRCLE ( 'NONE', #31575, 0.06509327318403745899 ) ;
#62960=CONICAL_SURFACE ( 'NONE', #56679, 0.1000000000000002554, 0.003490658503988666988 ) ;
#62961=CARTESIAN_POINT ( 'NONE',  ( 2.699999999999947331, 2.500000000000000000, -4.676537180435978769 ) ) ;
#62962=CARTESIAN_POINT ( 'NONE',  ( 13.74999999999989697, 2.500000000000000000, 2.857883832488649301 ) ) ;
#62963=EDGE_CURVE ( 'NONE', #16380, #110762, #41434, .T. ) ;
#62964=CARTESIAN_POINT ( 'NONE',  ( 6.849999999999929479, 12.50000000000000000, 6.776507416713035248 ) ) ;
#62965=VERTEX_POINT ( 'NONE', #89722 ) ;
#62966=VERTEX_POINT ( 'NONE', #28885 ) ;
#62967=FACE_BOUND ( 'NONE', #13712, .T. ) ;
#62968=VERTEX_POINT ( 'NONE', #98247 ) ;
#62969=ADVANCED_FACE ( 'NONE', ( #58350 ), #9237, .T. ) ;
#62970=CARTESIAN_POINT ( 'NONE',  ( 11.24999999999990763, 12.50000000000000000, 1.472243186433545459 ) ) ;
#62971=CARTESIAN_POINT ( 'NONE',  ( -11.05000000000000071, 2.500000000000000000, 6.941600689897073018 ) ) ;
#62972=DIRECTION ( 'NONE',  ( -4.274815082592931898E-19, -0.9999939076577903929, -0.003490651415223739937 ) ) ;
#62973=CARTESIAN_POINT ( 'NONE',  ( -1.450000000000035483, 2.500000000000000000, 1.918653347947321564 ) ) ;
#62975=CARTESIAN_POINT ( 'NONE',  ( -11.25000000000000178, 2.500000000000000000, -1.472243186433546125 ) ) ;
#62976=DIRECTION ( 'NONE',  ( 0.000000000000000000, 0.000000000000000000, 1.000000000000000000 ) ) ;
#62977=CARTESIAN_POINT ( 'NONE',  ( 6.249999999999930722, 12.50000000000000000, 7.253104124594885960 ) ) ;
#62978=EDGE_CURVE ( 'NONE', #47871, #89250, #1688, .T. ) ;
#62979=DIRECTION ( 'NONE',  ( 0.000000000000000000, 0.000000000000000000, 1.000000000000000000 ) ) ;
#62980=CARTESIAN_POINT ( 'NONE',  ( 6.049999999999934097, 2.500000000000000000, 6.148780366869520897 ) ) ;
#62981=CARTESIAN_POINT ( 'NONE',  ( -4.800000000000026468, 2.500000000000000000, -4.576537180435978236 ) ) ;
#62982=ORIENTED_EDGE ( 'NONE', *, *, #61884, .T. ) ;
#62983=EDGE_LOOP ( 'NONE', ( #58641, #88389 ) ) ;
#62984=EDGE_LOOP ( 'NONE', ( #129490, #110047 ) ) ;
#62985=DIRECTION ( 'NONE',  ( 0.000000000000000000, -0.000000000000000000, 1.000000000000000000 ) ) ;
#62986=ORIENTED_EDGE ( 'NONE', *, *, #94442, .T. ) ;
#62987=AXIS2_PLACEMENT_3D ( 'NONE', #16310, #56252, #57558 ) ;
#62988=DIRECTION ( 'NONE',  ( 0.000000000000000000, 0.000000000000000000, 1.000000000000000000 ) ) ;
#62989=CIRCLE ( 'NONE', #48317, 0.1000000000000002554 ) ;
#62990=AXIS2_PLACEMENT_3D ( 'NONE', #7459, #17259, #127891 ) ;
#62991=VERTEX_POINT ( 'NONE', #118531 ) ;
#62992=ORIENTED_EDGE ( 'NONE', *, *, #90423, .F. ) ;
#62993=VERTEX_POINT ( 'NONE', #68140 ) ;
#62994=CARTESIAN_POINT ( 'NONE',  ( 5.599999999999933031, 2.500000000000000000, 0.2464101615137735679 ) ) ;
#62995=VECTOR ( 'NONE', #24916, 1000.000000000000000 ) ;
#62996=DIRECTION ( 'NONE',  ( 0.000000000000000000, 0.000000000000000000, -1.000000000000000000 ) ) ;
#62998=ADVANCED_FACE ( 'NONE', ( #60294 ), #55969, .T. ) ;
#62999=LINE ( 'NONE', #93117, #70644 ) ;
#63000=DIRECTION ( 'NONE',  ( -4.274815082592931898E-19, -0.9999939076577903929, -0.003490651415223739937 ) ) ;
#63002=AXIS2_PLACEMENT_3D ( 'NONE', #105672, #4869, #25819 ) ;
#63003=LINE ( 'NONE', #13236, #24566 ) ;
#63004=ORIENTED_EDGE ( 'NONE', *, *, #14656, .T. ) ;
#63005=CARTESIAN_POINT ( 'NONE',  ( 1.449999999999950440, 12.50000000000000000, 6.148780366869520009 ) ) ;
#63006=ORIENTED_EDGE ( 'NONE', *, *, #96376, .F. ) ;
#63007=EDGE_CURVE ( 'NONE', #128448, #120284, #128388, .T. ) ;
#63008=ORIENTED_EDGE ( 'NONE', *, *, #121214, .T. ) ;
#63009=VERTEX_POINT ( 'NONE', #29521 ) ;
#63011=ADVANCED_FACE ( 'NONE', ( #18406 ), #116616, .T. ) ;
#63012=ORIENTED_EDGE ( 'NONE', *, *, #68458, .T. ) ;
#63014=EDGE_LOOP ( 'NONE', ( #84515, #78850, #81323, #53714 ) ) ;
#63015=EDGE_CURVE ( 'NONE', #67345, #22620, #26740, .T. ) ;
#63017=EDGE_CURVE ( 'NONE', #33832, #24400, #57698, .T. ) ;
#63019=CARTESIAN_POINT ( 'NONE',  ( -14.34999999999998543, 12.50000000000000000, -2.511473670974875727 ) ) ;
#63020=DIRECTION ( 'NONE',  ( -0.000000000000000000, 1.000000000000000000, -0.000000000000000000 ) ) ;
#63022=ADVANCED_FACE ( 'NONE', ( #108715 ), #72714, .T. ) ;
#63023=LINE ( 'NONE', #4091, #109429 ) ;
#63024=ADVANCED_FACE ( 'NONE', ( #110021 ), #83142, .T. ) ;
#63025=DIRECTION ( 'NONE',  ( 0.000000000000000000, 0.000000000000000000, 1.000000000000000000 ) ) ;
#63027=AXIS2_PLACEMENT_3D ( 'NONE', #85396, #125321, #95866 ) ;
#63028=ORIENTED_EDGE ( 'NONE', *, *, #70170, .T. ) ;
#63029=CARTESIAN_POINT ( 'NONE',  ( -6.450000000000017941, 12.50000000000000000, -6.841600689897077814 ) ) ;
#63030=EDGE_CURVE ( 'NONE', #128895, #110043, #12153, .T. ) ;
#63031=VERTEX_POINT ( 'NONE', #71355 ) ;
#63032=DIRECTION ( 'NONE',  ( 0.000000000000000000, -1.000000000000000000, 0.000000000000000000 ) ) ;
#63033=ORIENTED_EDGE ( 'NONE', *, *, #27831, .F. ) ;
#63034=EDGE_CURVE ( 'NONE', #16842, #123754, #81132, .T. ) ;
#63035=ORIENTED_EDGE ( 'NONE', *, *, #21666, .F. ) ;
#63037=EDGE_CURVE ( 'NONE', #6359, #66455, #120834, .T. ) ;
#63038=DIRECTION ( 'NONE',  ( 0.000000000000000000, -0.9999939076577903929, 0.003490651415223739937 ) ) ;
#63039=AXIS2_PLACEMENT_3D ( 'NONE', #106014, #26807, #125003 ) ;
#63040=AXIS2_PLACEMENT_3D ( 'NONE', #77679, #65932, #27951 ) ;
#63041=CARTESIAN_POINT ( 'NONE',  ( -3.950000000000028155, 2.500000000000000000, -6.941600689897077459 ) ) ;
#63042=ORIENTED_EDGE ( 'NONE', *, *, #28461, .T. ) ;
#63043=VERTEX_POINT ( 'NONE', #82499 ) ;
#63044=CARTESIAN_POINT ( 'NONE',  ( 3.749999999999940492, 2.500000000000000000, 2.857883832488649301 ) ) ;
#63045=CARTESIAN_POINT ( 'NONE',  ( 5.399999999999933742, 12.50000000000000000, -2.385244779468109755E-15 ) ) ;
#63046=FACE_OUTER_BOUND ( 'NONE', #78855, .T. ) ;
#63047=DIRECTION ( 'NONE',  ( -0.000000000000000000, 1.000000000000000000, -0.000000000000000000 ) ) ;
#63048=VECTOR ( 'NONE', #42314, 1000.000000000000000 ) ;
#63049=CONICAL_SURFACE ( 'NONE', #71432, 0.1000000000000002554, 0.003490658503988666988 ) ;
#63050=FACE_OUTER_BOUND ( 'NONE', #114319, .T. ) ;
#63051=EDGE_LOOP ( 'NONE', ( #90180, #110030, #66479, #27876 ) ) ;
#63052=CARTESIAN_POINT ( 'NONE',  ( -5.850000000000021849, 2.500000000000000000, -7.188010851410854052 ) ) ;
#63053=AXIS2_PLACEMENT_3D ( 'NONE', #17476, #50200, #19412 ) ;
#63054=AXIS2_PLACEMENT_3D ( 'NONE', #41547, #81458, #121362 ) ;
#63055=ORIENTED_EDGE ( 'NONE', *, *, #122697, .T. ) ;
#63056=DIRECTION ( 'NONE',  ( 0.000000000000000000, 0.000000000000000000, 1.000000000000000000 ) ) ;
#63057=FACE_OUTER_BOUND ( 'NONE', #74834, .T. ) ;
#63059=AXIS2_PLACEMENT_3D ( 'NONE', #69125, #59991, #70428 ) ;
#63061=DIRECTION ( 'NONE',  ( 0.000000000000000000, -0.9999939076577903929, 0.003490651415223739937 ) ) ;
#63062=FACE_OUTER_BOUND ( 'NONE', #122489, .T. ) ;
#63063=DIRECTION ( 'NONE',  ( -0.000000000000000000, 1.000000000000000000, -0.000000000000000000 ) ) ;
#63064=CARTESIAN_POINT ( 'NONE',  ( 4.149999999999938183, 2.500000000000000000, 2.165063509461097713 ) ) ;
#63065=ORIENTED_EDGE ( 'NONE', *, *, #123171, .F. ) ;
#63066=CARTESIAN_POINT ( 'NONE',  ( -12.89999999999999325, 2.500000000000000000, -3.537306695894647302 ) ) ;
#63067=EDGE_CURVE ( 'NONE', #118565, #56267, #51886, .T. ) ;
#63068=CARTESIAN_POINT ( 'NONE',  ( -6.650000000000014566, 2.500000000000000000, 1.472243186433545459 ) ) ;
#63069=DIRECTION ( 'NONE',  ( 0.000000000000000000, 0.000000000000000000, 1.000000000000000000 ) ) ;
#63070=EDGE_CURVE ( 'NONE', #43290, #850, #129177, .T. ) ;
#63071=ORIENTED_EDGE ( 'NONE', *, *, #23366, .T. ) ;
#63072=DIRECTION ( 'NONE',  ( -0.000000000000000000, -1.000000000000000000, -0.000000000000000000 ) ) ;
#63073=ORIENTED_EDGE ( 'NONE', *, *, #58574, .T. ) ;
#63074=ORIENTED_EDGE ( 'NONE', *, *, #39272, .T. ) ;
#63075=CARTESIAN_POINT ( 'NONE',  ( -9.800000000000006040, 2.500000000000000000, 0.3464101615137735735 ) ) ;
#63076=AXIS2_PLACEMENT_3D ( 'NONE', #88857, #120262, #80336 ) ;
#63077=AXIS2_PLACEMENT_3D ( 'NONE', #109054, #70451, #20708 ) ;
#63078=AXIS2_PLACEMENT_3D ( 'NONE', #125165, #44033, #75403 ) ;
#63079=ORIENTED_EDGE ( 'NONE', *, *, #49690, .F. ) ;
#63080=CARTESIAN_POINT ( 'NONE',  ( 20.80581321129333361, -0.6997403544382545526, -4.161084241360549107 ) ) ;
#63081=FACE_OUTER_BOUND ( 'NONE', #94274, .T. ) ;
#63082=CARTESIAN_POINT ( 'NONE',  ( -13.94999999999998685, 12.50000000000000000, -2.446380397790838046 ) ) ;
#63083=ORIENTED_EDGE ( 'NONE', *, *, #57259, .F. ) ;
#63084=CARTESIAN_POINT ( 'NONE',  ( -13.09999999999999254, 2.500000000000000000, 0.4464101615137777701 ) ) ;
#63085=AXIS2_PLACEMENT_3D ( 'NONE', #76686, #53348, #56386 ) ;
#63086=PLANE ( 'NONE',  #99734 ) ;
#63087=CIRCLE ( 'NONE', #17082, 0.06509327318403745899 ) ;
#63088=AXIS2_PLACEMENT_3D ( 'NONE', #113455, #12660, #51974 ) ;
#63089=VERTEX_POINT ( 'NONE', #1977 ) ;
#63090=CIRCLE ( 'NONE', #50566, 0.1000000000000000472 ) ;
#63091=ORIENTED_EDGE ( 'NONE', *, *, #43513, .T. ) ;
#63092=ORIENTED_EDGE ( 'NONE', *, *, #125327, .F. ) ;
#63093=DIRECTION ( 'NONE',  ( 0.000000000000000000, 1.000000000000000000, 0.000000000000000000 ) ) ;
#63094=LINE ( 'NONE', #82758, #73049 ) ;
#63095=CARTESIAN_POINT ( 'NONE',  ( -4.150000000000024336, 12.50000000000000000, -2.792790559304616504 ) ) ;
#63096=VERTEX_POINT ( 'NONE', #100814 ) ;
#63097=CARTESIAN_POINT ( 'NONE',  ( -1.250000000000001110, 2.500000000000000000, -6.495190528383302464 ) ) ;
#63098=CARTESIAN_POINT ( 'NONE',  ( 2.099999999999948574, 2.500000000000000000, 3.737306695894644371 ) ) ;
#63099=ORIENTED_EDGE ( 'NONE', *, *, #50726, .F. ) ;
#63100=CARTESIAN_POINT ( 'NONE',  ( -10.85000000000000142, 2.500000000000000000, -2.757883832488650100 ) ) ;
#63101=ADVANCED_FACE ( 'NONE', ( #13072 ), #16247, .T. ) ;
#63102=CARTESIAN_POINT ( 'NONE',  ( 9.599999999999917932, 12.50000000000000000, -0.6928203230275541413 ) ) ;
#63103=CARTESIAN_POINT ( 'NONE',  ( 1.649999999999951505, 12.50000000000000000, -2.857883832488653741 ) ) ;
#63104=CARTESIAN_POINT ( 'NONE',  ( 3.099999999999945022, 12.50000000000000000, -4.741630453620016006 ) ) ;
#63105=DIRECTION ( 'NONE',  ( -0.000000000000000000, -1.000000000000000000, -0.000000000000000000 ) ) ;
#63106=FACE_OUTER_BOUND ( 'NONE', #29690, .T. ) ;
#63107=DIRECTION ( 'NONE',  ( 0.000000000000000000, 1.000000000000000000, 0.000000000000000000 ) ) ;
#63108=EDGE_CURVE ( 'NONE', #33313, #78466, #118768, .T. ) ;
#63109=CIRCLE ( 'NONE', #125791, 0.1000000000000000056 ) ;
#63110=ORIENTED_EDGE ( 'NONE', *, *, #26404, .F. ) ;
#63111=ORIENTED_EDGE ( 'NONE', *, *, #46765, .F. ) ;
#63112=EDGE_LOOP ( 'NONE', ( #5551, #64776, #44288, #63099 ) ) ;
#63113=ORIENTED_EDGE ( 'NONE', *, *, #9962, .F. ) ;
#63114=DIRECTION ( 'NONE',  ( 0.000000000000000000, 0.000000000000000000, -1.000000000000000000 ) ) ;
#63115=LINE ( 'NONE', #114158, #97953 ) ;
#63116=EDGE_CURVE ( 'NONE', #17230, #85684, #102056, .T. ) ;
#63117=CARTESIAN_POINT ( 'NONE',  ( 7.299999999999926104, 2.500000000000000000, 4.676537180435972552 ) ) ;
#63118=ORIENTED_EDGE ( 'NONE', *, *, #96712, .F. ) ;
#63119=FACE_BOUND ( 'NONE', #71458, .T. ) ;
#63120=ADVANCED_FACE ( 'NONE', ( #22926 ), #93644, .T. ) ;
#63121=VECTOR ( 'NONE', #50217, 1000.000000000000000 ) ;
#63122=DIRECTION ( 'NONE',  ( -4.274815082592931898E-19, -0.9999939076577903929, -0.003490651415223739937 ) ) ;
#63123=FACE_OUTER_BOUND ( 'NONE', #57323, .T. ) ;
#63124=CIRCLE ( 'NONE', #29680, 0.09999999999999982514 ) ;
#63125=DIRECTION ( 'NONE',  ( 0.000000000000000000, 0.000000000000000000, -1.000000000000000000 ) ) ;
#63126=CARTESIAN_POINT ( 'NONE',  ( 13.29999999999989946, 2.500000000000000000, -2.385244779468109755E-15 ) ) ;
#63127=DIRECTION ( 'NONE',  ( -4.274815082592931898E-19, -0.9999939076577903929, -0.003490651415223739937 ) ) ;
#63128=DIRECTION ( 'NONE',  ( -4.274815082592931898E-19, -0.9999939076577903929, -0.003490651415223739937 ) ) ;
#63129=DIRECTION ( 'NONE',  ( 0.000000000000000000, 0.000000000000000000, 1.000000000000000000 ) ) ;
#63130=DIRECTION ( 'NONE',  ( 0.000000000000000000, 0.000000000000000000, 1.000000000000000000 ) ) ;
#63131=ADVANCED_FACE ( 'NONE', ( #92960 ), #3280, .T. ) ;
#63132=DIRECTION ( 'NONE',  ( 0.000000000000000000, 0.000000000000000000, -1.000000000000000000 ) ) ;
#63133=CIRCLE ( 'NONE', #90302, 0.06509327318403743123 ) ;
#63134=ORIENTED_EDGE ( 'NONE', *, *, #43425, .F. ) ;
#63135=CIRCLE ( 'NONE', #60981, 0.1000000000000002554 ) ;
#63136=ORIENTED_EDGE ( 'NONE', *, *, #68211, .T. ) ;
#63137=ORIENTED_EDGE ( 'NONE', *, *, #100229, .T. ) ;
#63138=EDGE_LOOP ( 'NONE', ( #45271, #23874, #73928, #2362 ) ) ;
#63139=AXIS2_PLACEMENT_3D ( 'NONE', #49929, #59090, #9335 ) ;
#63140=ORIENTED_EDGE ( 'NONE', *, *, #104529, .T. ) ;
#63141=AXIS2_PLACEMENT_3D ( 'NONE', #91183, #1502, #100996 ) ;
#63142=CIRCLE ( 'NONE', #98935, 0.06509327318403745899 ) ;
#63143=EDGE_LOOP ( 'NONE', ( #45475, #55202, #9640, #122650 ) ) ;
#63144=CARTESIAN_POINT ( 'NONE',  ( -8.150000000000012790, 2.500000000000000000, 1.918653347947321564 ) ) ;
#63145=ORIENTED_EDGE ( 'NONE', *, *, #65200, .T. ) ;
#63146=VERTEX_POINT ( 'NONE', #23559 ) ;
#63147=AXIS2_PLACEMENT_3D ( 'NONE', #36714, #77269, #117164 ) ;
#63148=AXIS2_PLACEMENT_3D ( 'NONE', #28192, #96916, #39328 ) ;
#63149=CARTESIAN_POINT ( 'NONE',  ( 9.399999999999915090, 12.50000000000000000, -4.611443907251939756 ) ) ;
#63150=DIRECTION ( 'NONE',  ( -0.000000000000000000, -1.000000000000000000, -0.000000000000000000 ) ) ;
#63151=PLANE ( 'NONE',  #46785 ) ;
#63152=EDGE_LOOP ( 'NONE', ( #24578, #5347 ) ) ;
#63153=DIRECTION ( 'NONE',  ( 0.000000000000000000, -0.000000000000000000, 1.000000000000000000 ) ) ;
#63154=ORIENTED_EDGE ( 'NONE', *, *, #86997, .T. ) ;
#63155=EDGE_CURVE ( 'NONE', #14213, #81272, #43479, .T. ) ;
#63156=ORIENTED_EDGE ( 'NONE', *, *, #18915, .F. ) ;
#63157=CARTESIAN_POINT ( 'NONE',  ( -12.09999999999999609, 12.50000000000000000, -3.637306695894647390 ) ) ;
#63158=DIRECTION ( 'NONE',  ( -0.000000000000000000, -1.000000000000000000, -0.000000000000000000 ) ) ;
#63159=ADVANCED_FACE ( 'NONE', ( #121753 ), #5879, .T. ) ;
#63160=ORIENTED_EDGE ( 'NONE', *, *, #23880, .T. ) ;
#63161=ORIENTED_EDGE ( 'NONE', *, *, #127465, .F. ) ;
#63163=LINE ( 'NONE', #125310, #92356 ) ;
#63164=DIRECTION ( 'NONE',  ( 0.000000000000000000, 1.000000000000000000, 0.000000000000000000 ) ) ;
#63165=DIRECTION ( 'NONE',  ( -0.000000000000000000, -1.000000000000000000, -0.000000000000000000 ) ) ;
#63167=CARTESIAN_POINT ( 'NONE',  ( -3.300000000000028244, 2.500000000000000000, 4.430127018922196847 ) ) ;
#63168=AXIS2_PLACEMENT_3D ( 'NONE', #89705, #100177, #31 ) ;
#63169=ADVANCED_FACE ( 'NONE', ( #111955 ), #70729, .T. ) ;
#63170=VECTOR ( 'NONE', #118554, 1000.000000000000000 ) ;
#63171=EDGE_CURVE ( 'NONE', #118, #54102, #5788, .T. ) ;
#63172=FACE_OUTER_BOUND ( 'NONE', #115692, .T. ) ;
#63173=ADVANCED_FACE ( 'NONE', ( #101487 ), #95705, .T. ) ;
#63174=EDGE_CURVE ( 'NONE', #84243, #14399, #54310, .T. ) ;
#63175=ORIENTED_EDGE ( 'NONE', *, *, #50547, .F. ) ;
#63176=CARTESIAN_POINT ( 'NONE',  ( 8.920123399827042832, -2.500000000000000000, 8.410822907074534172 ) ) ;
#63177=CIRCLE ( 'NONE', #31792, 0.06509327318403745899 ) ;
#63178=CIRCLE ( 'NONE', #48513, 0.09999999999999999167 ) ;
#63179=ORIENTED_EDGE ( 'NONE', *, *, #72059, .T. ) ;
#63180=CARTESIAN_POINT ( 'NONE',  ( 7.899999999999923084, 12.50000000000000000, -0.6928203230275542523 ) ) ;
#63181=CIRCLE ( 'NONE', #111272, 0.06509327318403745899 ) ;
#63182=EDGE_CURVE ( 'NONE', #24862, #97815, #127103, .T. ) ;
#63183=EDGE_LOOP ( 'NONE', ( #13850, #85641, #26512, #46206 ) ) ;
#63184=CARTESIAN_POINT ( 'NONE',  ( 7.949999999999925571, 12.50000000000000000, -6.495190528383302464 ) ) ;
#63186=CIRCLE ( 'NONE', #81951, 0.1000000000000000472 ) ;
#63188=DIRECTION ( 'NONE',  ( -4.274815082592931898E-19, -0.9999939076577903929, -0.003490651415223739937 ) ) ;
#63189=DIRECTION ( 'NONE',  ( 0.000000000000000000, 0.000000000000000000, -1.000000000000000000 ) ) ;
#63191=EDGE_CURVE ( 'NONE', #39789, #118565, #44486, .T. ) ;
#63192=AXIS2_PLACEMENT_3D ( 'NONE', #126792, #113755, #124856 ) ;
#63193=DIRECTION ( 'NONE',  ( 0.000000000000000000, -0.000000000000000000, 1.000000000000000000 ) ) ;
#63194=DIRECTION ( 'NONE',  ( 0.000000000000000000, 0.000000000000000000, -1.000000000000000000 ) ) ;
#63195=ORIENTED_EDGE ( 'NONE', *, *, #5321, .F. ) ;
#63196=ORIENTED_EDGE ( 'NONE', *, *, #8158, .T. ) ;
#63197=ORIENTED_EDGE ( 'NONE', *, *, #1862, .F. ) ;
#63198=PLANE ( 'NONE',  #12048 ) ;
#63199=CARTESIAN_POINT ( 'NONE',  ( -13.34999999999999076, 2.500000000000000000, -2.957883832488651610 ) ) ;
#63201=DIRECTION ( 'NONE',  ( 0.000000000000000000, 0.000000000000000000, 1.000000000000000000 ) ) ;
#63202=DIRECTION ( 'NONE',  ( 0.000000000000000000, -0.9999939076577903929, 0.003490651415223739937 ) ) ;
#63203=CARTESIAN_POINT ( 'NONE',  ( 5.649999999999934630, 2.500000000000000000, 6.248780366869521430 ) ) ;
#63205=VECTOR ( 'NONE', #9456, 1000.000000000000000 ) ;
#63206=ORIENTED_EDGE ( 'NONE', *, *, #16603, .F. ) ;
#63207=CARTESIAN_POINT ( 'NONE',  ( -6.249999999999984901, 2.500000000000000000, -6.595190528383302109 ) ) ;
#63208=ORIENTED_EDGE ( 'NONE', *, *, #37308, .F. ) ;
#63209=DIRECTION ( 'NONE',  ( 0.000000000000000000, -0.000000000000000000, 1.000000000000000000 ) ) ;
#63210=DIRECTION ( 'NONE',  ( -0.000000000000000000, -1.000000000000000000, -0.000000000000000000 ) ) ;
#63211=CARTESIAN_POINT ( 'NONE',  ( 5.649999999999934630, 12.50000000000000000, -2.511473670974877948 ) ) ;
#63212=CARTESIAN_POINT ( 'NONE',  ( 7.699999999999925571, 12.50000000000000000, -4.676537180435978769 ) ) ;
#63214=EDGE_LOOP ( 'NONE', ( #33500, #113628 ) ) ;
#63215=DIRECTION ( 'NONE',  ( -4.274815082592931898E-19, -0.9999939076577903929, -0.003490651415223739937 ) ) ;
#63216=VECTOR ( 'NONE', #80041, 1000.000000000000000 ) ;
#63217=AXIS2_PLACEMENT_3D ( 'NONE', #20557, #108910, #100406 ) ;
#63218=EDGE_CURVE ( 'NONE', #60850, #65138, #14998, .T. ) ;
#63219=DIRECTION ( 'NONE',  ( -4.274815082592931898E-19, -0.9999939076577903929, -0.003490651415223739937 ) ) ;
#63220=DIRECTION ( 'NONE',  ( -0.000000000000000000, -1.000000000000000000, -0.000000000000000000 ) ) ;
#63221=ORIENTED_EDGE ( 'NONE', *, *, #13698, .F. ) ;
#63222=AXIS2_PLACEMENT_3D ( 'NONE', #14442, #103494, #13800 ) ;
#63223=ORIENTED_EDGE ( 'NONE', *, *, #19870, .F. ) ;
#63224=CARTESIAN_POINT ( 'NONE',  ( -12.09999999999999609, 2.500000000000000000, -0.5928203230275500557 ) ) ;
#63225=CONICAL_SURFACE ( 'NONE', #29777, 0.1000000000000002554, 0.003490658503988666988 ) ;
#63226=ADVANCED_FACE ( 'NONE', ( #84411 ), #124985, .T. ) ;
#63227=ORIENTED_EDGE ( 'NONE', *, *, #93893, .T. ) ;
#63228=VECTOR ( 'NONE', #106631, 1000.000000000000000 ) ;
#63229=AXIS2_PLACEMENT_3D ( 'NONE', #81216, #30839, #51754 ) ;
#63230=ORIENTED_EDGE ( 'NONE', *, *, #20478, .F. ) ;
#63231=CONICAL_SURFACE ( 'NONE', #71547, 0.1000000000000000056, 0.003490658503988666988 ) ;
#63232=DIRECTION ( 'NONE',  ( 0.000000000000000000, 0.000000000000000000, 1.000000000000000000 ) ) ;
#63233=VECTOR ( 'NONE', #75183, 1000.000000000000000 ) ;
#63234=ORIENTED_EDGE ( 'NONE', *, *, #18645, .T. ) ;
#63235=DIRECTION ( 'NONE',  ( 0.000000000000000000, -0.9999939076577903929, 0.003490651415223739937 ) ) ;
#63236=DIRECTION ( 'NONE',  ( 0.000000000000000000, -0.000000000000000000, 1.000000000000000000 ) ) ;
#63237=DIRECTION ( 'NONE',  ( 0.000000000000000000, 1.000000000000000000, 0.000000000000000000 ) ) ;
#63238=EDGE_LOOP ( 'NONE', ( #123870, #16168 ) ) ;
#63239=CIRCLE ( 'NONE', #44363, 0.06509327318403745899 ) ;
#63240=CARTESIAN_POINT ( 'NONE',  ( -1.850000000000033840, 2.500000000000000000, 6.048780366869521252 ) ) ;
#63241=DIRECTION ( 'NONE',  ( 0.000000000000000000, 1.000000000000000000, 0.000000000000000000 ) ) ;
#63243=LINE ( 'NONE', #81589, #79842 ) ;
#63244=DIRECTION ( 'NONE',  ( -0.000000000000000000, 1.000000000000000000, -0.000000000000000000 ) ) ;
#63245=ORIENTED_EDGE ( 'NONE', *, *, #14034, .T. ) ;
#63246=ORIENTED_EDGE ( 'NONE', *, *, #4510, .F. ) ;
#63247=ORIENTED_EDGE ( 'NONE', *, *, #127753, .F. ) ;
#63248=ORIENTED_EDGE ( 'NONE', *, *, #50395, .T. ) ;
#63249=DIRECTION ( 'NONE',  ( 0.000000000000000000, 0.000000000000000000, -1.000000000000000000 ) ) ;
#63250=DIRECTION ( 'NONE',  ( 0.000000000000000000, 0.000000000000000000, 1.000000000000000000 ) ) ;
#63252=FACE_BOUND ( 'NONE', #5187, .T. ) ;
#63253=VERTEX_POINT ( 'NONE', #35962 ) ;
#63255=CARTESIAN_POINT ( 'NONE',  ( -12.09999999999999609, 2.500000000000000000, -0.09999999999999827083 ) ) ;
#63257=EDGE_CURVE ( 'NONE', #103010, #115225, #114507, .T. ) ;
#63258=AXIS2_PLACEMENT_3D ( 'NONE', #3896, #43852, #24194 ) ;
#63259=DIRECTION ( 'NONE',  ( 0.000000000000000000, 0.000000000000000000, 1.000000000000000000 ) ) ;
#63260=CARTESIAN_POINT ( 'NONE',  ( -11.44999999999999751, 2.500000000000000000, 1.718653347947321386 ) ) ;
#63261=DIRECTION ( 'NONE',  ( 0.000000000000000000, 0.000000000000000000, 1.000000000000000000 ) ) ;
#63262=EDGE_CURVE ( 'NONE', #25742, #47551, #30970, .T. ) ;
#63263=CIRCLE ( 'NONE', #56984, 0.06509327318403745899 ) ;
#63264=DIRECTION ( 'NONE',  ( -0.000000000000000000, -1.000000000000000000, -0.000000000000000000 ) ) ;
#63265=AXIS2_PLACEMENT_3D ( 'NONE', #6196, #75585, #15369 ) ;
#63266=ORIENTED_EDGE ( 'NONE', *, *, #29726, .T. ) ;
#63267=VERTEX_POINT ( 'NONE', #94880 ) ;
#63268=EDGE_LOOP ( 'NONE', ( #75121, #25935 ) ) ;
#63269=VERTEX_POINT ( 'NONE', #5192 ) ;
#63270=ORIENTED_EDGE ( 'NONE', *, *, #106007, .F. ) ;
#63272=CONICAL_SURFACE ( 'NONE', #36192, 0.09999999999999982514, 0.003490658503988666988 ) ;
#63273=EDGE_CURVE ( 'NONE', #43734, #82187, #66698, .T. ) ;
#63274=FACE_OUTER_BOUND ( 'NONE', #100095, .T. ) ;
#63275=VERTEX_POINT ( 'NONE', #6458 ) ;
#63276=FACE_BOUND ( 'NONE', #107242, .T. ) ;
#63277=ADVANCED_FACE ( 'NONE', ( #47083 ), #108394, .T. ) ;
#63278=AXIS2_PLACEMENT_3D ( 'NONE', #7642, #27284, #128748 ) ;
#63279=CARTESIAN_POINT ( 'NONE',  ( 8.099999999999923261, 2.500000000000000000, -4.676537180435978769 ) ) ;
#63280=EDGE_CURVE ( 'NONE', #123030, #35299, #114650, .T. ) ;
#63281=VERTEX_POINT ( 'NONE', #15653 ) ;
#63282=DIRECTION ( 'NONE',  ( -0.000000000000000000, 1.000000000000000000, -0.000000000000000000 ) ) ;
#63283=DIRECTION ( 'NONE',  ( 0.000000000000000000, 0.000000000000000000, 1.000000000000000000 ) ) ;
#63284=EDGE_CURVE ( 'NONE', #5264, #17021, #25478, .T. ) ;
#63285=CARTESIAN_POINT ( 'NONE',  ( -2.900000000000030553, 2.500000000000000000, 5.122947341949749323 ) ) ;
#63286=VERTEX_POINT ( 'NONE', #104683 ) ;
#63287=ORIENTED_EDGE ( 'NONE', *, *, #94241, .T. ) ;
#63288=VERTEX_POINT ( 'NONE', #24211 ) ;
#63289=ORIENTED_EDGE ( 'NONE', *, *, #84249, .T. ) ;
#63290=DIRECTION ( 'NONE',  ( 0.000000000000000000, 1.000000000000000000, 0.000000000000000000 ) ) ;
#63291=DIRECTION ( 'NONE',  ( -4.274815082592931898E-19, -0.9999939076577903929, -0.003490651415223739937 ) ) ;
#63292=CARTESIAN_POINT ( 'NONE',  ( 6.849999999999930367, 12.50000000000000000, -6.083687093685488989 ) ) ;
#63293=EDGE_LOOP ( 'NONE', ( #127610, #124500, #109224, #66908 ) ) ;
#63294=CARTESIAN_POINT ( 'NONE',  ( 10.19999999999991047, 2.500000000000000000, 4.676537180435972552 ) ) ;
#63295=CONICAL_SURFACE ( 'NONE', #50781, 0.1000000000000002554, 0.003490658503988666988 ) ;
#63296=VECTOR ( 'NONE', #18018, 1000.000000000000000 ) ;
#63297=CIRCLE ( 'NONE', #13104, 0.06509327318403745899 ) ;
#63298=DIRECTION ( 'NONE',  ( 0.000000000000000000, -0.000000000000000000, 1.000000000000000000 ) ) ;
#63299=DIRECTION ( 'NONE',  ( 0.000000000000000000, 1.000000000000000000, 0.000000000000000000 ) ) ;
#63301=ORIENTED_EDGE ( 'NONE', *, *, #95996, .T. ) ;
#63302=CARTESIAN_POINT ( 'NONE',  ( -1.850000000000033840, 12.50000000000000000, 2.511473670974873507 ) ) ;
#63303=AXIS2_PLACEMENT_3D ( 'NONE', #125692, #66779, #115212 ) ;
#63304=ORIENTED_EDGE ( 'NONE', *, *, #68057, .T. ) ;
#63305=DIRECTION ( 'NONE',  ( 0.000000000000000000, 0.000000000000000000, 1.000000000000000000 ) ) ;
#63306=VECTOR ( 'NONE', #67999, 1000.000000000000000 ) ;
#63307=AXIS2_PLACEMENT_3D ( 'NONE', #51879, #92433, #74087 ) ;
#63308=EDGE_LOOP ( 'NONE', ( #87432, #110618, #53641, #22498 ) ) ;
#63309=ORIENTED_EDGE ( 'NONE', *, *, #115511, .F. ) ;
#63310=DIRECTION ( 'NONE',  ( -4.274815082592931898E-19, -0.9999939076577903929, -0.003490651415223739937 ) ) ;
#63312=DIRECTION ( 'NONE',  ( 0.000000000000000000, 1.000000000000000000, 0.000000000000000000 ) ) ;
#63313=DIRECTION ( 'NONE',  ( 0.000000000000000000, 1.000000000000000000, 0.000000000000000000 ) ) ;
#63314=DIRECTION ( 'NONE',  ( -0.000000000000000000, 1.000000000000000000, -0.000000000000000000 ) ) ;
#63315=VECTOR ( 'NONE', #111876, 1000.000000000000000 ) ;
#63316=ORIENTED_EDGE ( 'NONE', *, *, #110213, .F. ) ;
#63317=EDGE_LOOP ( 'NONE', ( #90031, #38068 ) ) ;
#63318=DIRECTION ( 'NONE',  ( 0.000000000000000000, 0.000000000000000000, -1.000000000000000000 ) ) ;
#63319=FACE_OUTER_BOUND ( 'NONE', #10024, .T. ) ;
#63320=CIRCLE ( 'NONE', #84239, 0.1000000000000000472 ) ;
#63321=CIRCLE ( 'NONE', #50815, 0.1000000000000000056 ) ;
#63322=AXIS2_PLACEMENT_3D ( 'NONE', #12424, #112582, #1319 ) ;
#63324=EDGE_CURVE ( 'NONE', #48575, #74213, #1774, .T. ) ;
#63325=ORIENTED_EDGE ( 'NONE', *, *, #17763, .F. ) ;
#63326=ORIENTED_EDGE ( 'NONE', *, *, #113129, .T. ) ;
#63327=EDGE_CURVE ( 'NONE', #18996, #55517, #120917, .T. ) ;
#63329=VECTOR ( 'NONE', #32555, 1000.000000000000000 ) ;
#63331=EDGE_CURVE ( 'NONE', #8330, #124875, #26835, .T. ) ;
#63332=ORIENTED_EDGE ( 'NONE', *, *, #67265, .F. ) ;
#63333=CARTESIAN_POINT ( 'NONE',  ( -4.350000000000023626, 12.50000000000000000, -2.511473670974877948 ) ) ;
#63334=FACE_OUTER_BOUND ( 'NONE', #126490, .T. ) ;
#63335=CARTESIAN_POINT ( 'NONE',  ( 0.7999999999999612976, 12.50000000000000000, 0.06509327318403732021 ) ) ;
#63336=ORIENTED_EDGE ( 'NONE', *, *, #19982, .T. ) ;
#63337=CONICAL_SURFACE ( 'NONE', #2673, 0.1000000000000002554, 0.003490658503988666988 ) ;
#63338=CARTESIAN_POINT ( 'NONE',  ( -5.000000000000022204, 2.500000000000000000, -0.7928203230275542301 ) ) ;
#63339=CARTESIAN_POINT ( 'NONE',  ( 11.64999999999990443, 2.500000000000000000, -5.902370205355750521 ) ) ;
#63340=ADVANCED_FACE ( 'NONE', ( #76535 ), #77005, .T. ) ;
#63341=CARTESIAN_POINT ( 'NONE',  ( -13.29999999999998828, 2.500000000000000000, 4.230127018922196669 ) ) ;
#63342=CARTESIAN_POINT ( 'NONE',  ( -11.64999999999999680, 12.50000000000000000, 5.737276932171707422 ) ) ;
#63343=DIRECTION ( 'NONE',  ( 0.000000000000000000, 0.000000000000000000, -1.000000000000000000 ) ) ;
#63344=EDGE_LOOP ( 'NONE', ( #68027, #63028 ) ) ;
#63345=EDGE_CURVE ( 'NONE', #98888, #122658, #68685, .T. ) ;
#63346=LINE ( 'NONE', #33878, #90583 ) ;
#63347=EDGE_CURVE ( 'NONE', #85021, #114482, #79174, .T. ) ;
#63348=CARTESIAN_POINT ( 'NONE',  ( 4.399999999999940847, 12.50000000000000000, -4.676537180435977881 ) ) ;
#63349=ORIENTED_EDGE ( 'NONE', *, *, #3558, .F. ) ;
#63350=ORIENTED_EDGE ( 'NONE', *, *, #25814, .T. ) ;
#63351=CONICAL_SURFACE ( 'NONE', #6878, 0.1000000000000002554, 0.003490658503988666988 ) ;
#63353=CARTESIAN_POINT ( 'NONE',  ( -13.74999999999998757, 12.50000000000000000, 1.472243186433549456 ) ) ;
#63354=CARTESIAN_POINT ( 'NONE',  ( -9.600000000000008527, 2.500000000000000000, -4.922947341949749145 ) ) ;
#63355=DIRECTION ( 'NONE',  ( -4.274815082592931898E-19, -0.9999939076577903929, -0.003490651415223739937 ) ) ;
#63356=CARTESIAN_POINT ( 'NONE',  ( 12.89999999999989910, 12.50000000000000000, 0.7579135962115869374 ) ) ;
#63357=VECTOR ( 'NONE', #49562, 1000.000000000000000 ) ;
#63358=DIRECTION ( 'NONE',  ( -0.000000000000000000, -1.000000000000000000, -0.000000000000000000 ) ) ;
#63359=CARTESIAN_POINT ( 'NONE',  ( -8.100000000000010303, 12.50000000000000000, 4.048810130592458201 ) ) ;
#63360=CIRCLE ( 'NONE', #42442, 0.06509327318403745899 ) ;
#63361=DIRECTION ( 'NONE',  ( -0.000000000000000000, 1.000000000000000000, -0.000000000000000000 ) ) ;
#63362=DIRECTION ( 'NONE',  ( 0.000000000000000000, 1.000000000000000000, 0.000000000000000000 ) ) ;
#63363=CARTESIAN_POINT ( 'NONE',  ( -8.100000000000013856, 2.500000000000000000, 0.3464101615137736845 ) ) ;
#63364=CONICAL_SURFACE ( 'NONE', #88477, 0.1000000000000000056, 0.003490658503988666988 ) ;
#63365=AXIS2_PLACEMENT_3D ( 'NONE', #45503, #44186, #84109 ) ;
#63366=DIRECTION ( 'NONE',  ( 0.000000000000000000, 0.000000000000000000, 1.000000000000000000 ) ) ;
#63367=ORIENTED_EDGE ( 'NONE', *, *, #98583, .F. ) ;
#63368=VECTOR ( 'NONE', #7984, 1000.000000000000000 ) ;
#63369=EDGE_LOOP ( 'NONE', ( #110399, #21462, #113468, #123207 ) ) ;
#63370=CIRCLE ( 'NONE', #48798, 0.06509327318403745899 ) ;
#63371=ORIENTED_EDGE ( 'NONE', *, *, #1802, .F. ) ;
#63372=CIRCLE ( 'NONE', #21599, 0.06509327318403743123 ) ;
#63373=CONICAL_SURFACE ( 'NONE', #75972, 0.09999999999999999167, 0.003490658503988666988 ) ;
#63374=ORIENTED_EDGE ( 'NONE', *, *, #8004, .T. ) ;
#63375=CARTESIAN_POINT ( 'NONE',  ( -11.64999999999999680, 12.50000000000000000, 6.430097255199259010 ) ) ;
#63376=FACE_OUTER_BOUND ( 'NONE', #65602, .T. ) ;
#63377=AXIS2_PLACEMENT_3D ( 'NONE', #85878, #117258, #115997 ) ;
#63378=ORIENTED_EDGE ( 'NONE', *, *, #85536, .F. ) ;
#63379=DIRECTION ( 'NONE',  ( 1.000000000000000000, 0.000000000000000000, -0.000000000000000000 ) ) ;
#63380=DIRECTION ( 'NONE',  ( -0.000000000000000000, 1.000000000000000000, -0.000000000000000000 ) ) ;
#63381=LINE ( 'NONE', #103309, #28684 ) ;
#63382=VERTEX_POINT ( 'NONE', #80243 ) ;
#63383=DIRECTION ( 'NONE',  ( 0.000000000000000000, 1.000000000000000000, 0.000000000000000000 ) ) ;
#63384=VECTOR ( 'NONE', #68871, 1000.000000000000000 ) ;
#63385=DIRECTION ( 'NONE',  ( -0.000000000000000000, -1.000000000000000000, -0.000000000000000000 ) ) ;
#63386=VERTEX_POINT ( 'NONE', #129364 ) ;
#63387=EDGE_CURVE ( 'NONE', #51338, #47295, #41622, .T. ) ;
#63388=EDGE_LOOP ( 'NONE', ( #126211, #54962, #60325, #113350 ) ) ;
#63389=EDGE_LOOP ( 'NONE', ( #17306, #82514, #123580, #38224 ) ) ;
#63390=VERTEX_POINT ( 'NONE', #117076 ) ;
#63391=CARTESIAN_POINT ( 'NONE',  ( 5.649999999999934630, 2.500000000000000000, 6.048780366869521252 ) ) ;
#63392=VECTOR ( 'NONE', #75773, 1000.000000000000000 ) ;
#63393=LINE ( 'NONE', #14895, #11148 ) ;
#63394=DIRECTION ( 'NONE',  ( 0.000000000000000000, 0.000000000000000000, 1.000000000000000000 ) ) ;
#63395=CIRCLE ( 'NONE', #92637, 0.1000000000000002554 ) ;
#63396=DIRECTION ( 'NONE',  ( -0.000000000000000000, -1.000000000000000000, -0.000000000000000000 ) ) ;
#63397=AXIS2_PLACEMENT_3D ( 'NONE', #31859, #61321, #122814 ) ;
#63398=VERTEX_POINT ( 'NONE', #90037 ) ;
#63399=CARTESIAN_POINT ( 'NONE',  ( -5.650000000000019895, 12.50000000000000000, 6.841600689897072485 ) ) ;
#63400=ORIENTED_EDGE ( 'NONE', *, *, #109843, .F. ) ;
#63401=LINE ( 'NONE', #12355, #64265 ) ;
#63402=LINE ( 'NONE', #2522, #99919 ) ;
#63403=LINE ( 'NONE', #94145, #71381 ) ;
#63404=FACE_OUTER_BOUND ( 'NONE', #71335, .T. ) ;
#63405=AXIS2_PLACEMENT_3D ( 'NONE', #107777, #19379, #59995 ) ;
#63406=AXIS2_PLACEMENT_3D ( 'NONE', #28543, #29204, #126746 ) ;
#63407=EDGE_LOOP ( 'NONE', ( #57974, #39879 ) ) ;
#63408=CIRCLE ( 'NONE', #121994, 0.06509327318403745899 ) ;
#63409=EDGE_LOOP ( 'NONE', ( #12145, #15414, #29121, #66028 ) ) ;
#63410=EDGE_LOOP ( 'NONE', ( #33952, #25166, #103806, #70565 ) ) ;
#63411=DIRECTION ( 'NONE',  ( 0.000000000000000000, 0.000000000000000000, -1.000000000000000000 ) ) ;
#63412=LINE ( 'NONE', #53601, #106227 ) ;
#63413=DIRECTION ( 'NONE',  ( -0.000000000000000000, -1.000000000000000000, -0.000000000000000000 ) ) ;
#63414=FACE_BOUND ( 'NONE', #73481, .T. ) ;
#63415=CARTESIAN_POINT ( 'NONE',  ( 5.849999999999933920, 2.500000000000000000, -2.165063509461101710 ) ) ;
#63416=DIRECTION ( 'NONE',  ( -0.000000000000000000, -1.000000000000000000, -0.000000000000000000 ) ) ;
#63417=CARTESIAN_POINT ( 'NONE',  ( 10.59999999999990905, 2.500000000000000000, 4.776537180435972196 ) ) ;
#63418=AXIS2_PLACEMENT_3D ( 'NONE', #1577, #121352, #52614 ) ;
#63420=AXIS2_PLACEMENT_3D ( 'NONE', #42397, #100645, #1170 ) ;
#63421=FACE_OUTER_BOUND ( 'NONE', #10765, .T. ) ;
#63422=DIRECTION ( 'NONE',  ( 0.000000000000000000, 1.000000000000000000, 0.000000000000000000 ) ) ;
#63423=AXIS2_PLACEMENT_3D ( 'NONE', #15443, #74385, #85493 ) ;
#63424=DIRECTION ( 'NONE',  ( -0.000000000000000000, 1.000000000000000000, -0.000000000000000000 ) ) ;
#63425=ORIENTED_EDGE ( 'NONE', *, *, #21162, .T. ) ;
#63426=EDGE_CURVE ( 'NONE', #39960, #7581, #104194, .T. ) ;
#63427=DIRECTION ( 'NONE',  ( 0.000000000000000000, -0.9999939076577903929, 0.003490651415223739937 ) ) ;
#63428=ORIENTED_EDGE ( 'NONE', *, *, #35685, .F. ) ;
#63429=VERTEX_POINT ( 'NONE', #126927 ) ;
#63431=LINE ( 'NONE', #113827, #19307 ) ;
#63432=FACE_BOUND ( 'NONE', #68418, .T. ) ;
#63433=ADVANCED_FACE ( 'NONE', ( #79593 ), #67316, .T. ) ;
#63434=CARTESIAN_POINT ( 'NONE',  ( 1.049999999999954525, 2.500000000000000000, 1.818653347947321475 ) ) ;
#63435=ADVANCED_FACE ( 'NONE', ( #100510 ), #47770, .T. ) ;
#63436=EDGE_CURVE ( 'NONE', #97069, #121109, #70748, .T. ) ;
#63437=AXIS2_PLACEMENT_3D ( 'NONE', #75241, #115809, #37269 ) ;
#63438=ORIENTED_EDGE ( 'NONE', *, *, #35735, .T. ) ;
#63439=CARTESIAN_POINT ( 'NONE',  ( 26.76314062975745856, 1.072173157153399226, 4.440523076943353686 ) ) ;
#63440=CIRCLE ( 'NONE', #65482, 0.06509327318403745899 ) ;
#63441=EDGE_CURVE ( 'NONE', #72699, #31251, #119502, .T. ) ;
#63442=ADVANCED_FACE ( 'NONE', ( #40324 ), #51978, .T. ) ;
#63443=DIRECTION ( 'NONE',  ( 0.000000000000000000, 0.000000000000000000, -1.000000000000000000 ) ) ;
#63444=ADVANCED_FACE ( 'NONE', ( #59982 ), #101815, .T. ) ;
#63445=VERTEX_POINT ( 'NONE', #10208 ) ;
#63446=CARTESIAN_POINT ( 'NONE',  ( 6.849999999999929479, 12.50000000000000000, 6.148780366869520009 ) ) ;
#63448=AXIS2_PLACEMENT_3D ( 'NONE', #60667, #52133, #100567 ) ;
#63449=CIRCLE ( 'NONE', #105304, 0.06509327318403745899 ) ;
#63450=AXIS2_PLACEMENT_3D ( 'NONE', #45739, #35284, #55557 ) ;
#63452=ORIENTED_EDGE ( 'NONE', *, *, #54719, .F. ) ;
#63453=DIRECTION ( 'NONE',  ( -0.000000000000000000, -1.000000000000000000, -0.000000000000000000 ) ) ;
#63454=DIRECTION ( 'NONE',  ( 0.000000000000000000, 0.000000000000000000, -1.000000000000000000 ) ) ;
#63455=EDGE_CURVE ( 'NONE', #106728, #71667, #97455, .T. ) ;
#63456=AXIS2_PLACEMENT_3D ( 'NONE', #40706, #82550, #72721 ) ;
#63457=AXIS2_PLACEMENT_3D ( 'NONE', #111681, #122784, #82217 ) ;
#63458=ORIENTED_EDGE ( 'NONE', *, *, #63561, .F. ) ;
#63459=CONICAL_SURFACE ( 'NONE', #23760, 0.09999999999999999167, 0.003490658503988666988 ) ;
#63460=CARTESIAN_POINT ( 'NONE',  ( -11.44999999999999751, 2.500000000000000000, 6.841600689897072485 ) ) ;
#63461=DIRECTION ( 'NONE',  ( -0.000000000000000000, 1.000000000000000000, -0.000000000000000000 ) ) ;
#63462=FACE_OUTER_BOUND ( 'NONE', #5845, .T. ) ;
#63463=AXIS2_PLACEMENT_3D ( 'NONE', #118215, #59326, #99234 ) ;
#63464=AXIS2_PLACEMENT_3D ( 'NONE', #50461, #81226, #119853 ) ;
#63465=ORIENTED_EDGE ( 'NONE', *, *, #968, .F. ) ;
#63466=ORIENTED_EDGE ( 'NONE', *, *, #59161, .T. ) ;
#63467=DIRECTION ( 'NONE',  ( 0.000000000000000000, 0.000000000000000000, -1.000000000000000000 ) ) ;
#63468=ORIENTED_EDGE ( 'NONE', *, *, #22518, .T. ) ;
#63469=DIRECTION ( 'NONE',  ( 0.000000000000000000, -0.000000000000000000, 1.000000000000000000 ) ) ;
#63470=CARTESIAN_POINT ( 'NONE',  ( 10.84999999999991260, 2.500000000000000000, 7.188010851410848723 ) ) ;
#63471=ORIENTED_EDGE ( 'NONE', *, *, #42787, .T. ) ;
#63472=CARTESIAN_POINT ( 'NONE',  ( 9.149999999999918643, 2.500000000000000000, 2.165063509461097713 ) ) ;
#63473=CARTESIAN_POINT ( 'NONE',  ( -6.900000000000015454, 2.500000000000000000, 4.776537180435972196 ) ) ;
#63474=DIRECTION ( 'NONE',  ( 0.000000000000000000, 0.000000000000000000, 1.000000000000000000 ) ) ;
#63476=DIRECTION ( 'NONE',  ( -0.000000000000000000, -1.000000000000000000, -0.000000000000000000 ) ) ;
#63477=AXIS2_PLACEMENT_3D ( 'NONE', #21718, #53113, #14449 ) ;
#63479=EDGE_LOOP ( 'NONE', ( #39465, #43275, #59565, #22126 ) ) ;
#63480=CARTESIAN_POINT ( 'NONE',  ( 10.39999999999990976, 2.500000000000000000, 4.330127018922196314 ) ) ;
#63481=FACE_OUTER_BOUND ( 'NONE', #16649, .T. ) ;
#63482=EDGE_CURVE ( 'NONE', #69018, #123444, #20577, .T. ) ;
#63483=ORIENTED_EDGE ( 'NONE', *, *, #83843, .F. ) ;
#63484=ORIENTED_EDGE ( 'NONE', *, *, #13034, .T. ) ;
#63485=ORIENTED_EDGE ( 'NONE', *, *, #117149, .T. ) ;
#63486=EDGE_CURVE ( 'NONE', #27243, #67262, #56061, .T. ) ;
#63487=DIRECTION ( 'NONE',  ( 0.000000000000000000, -0.000000000000000000, 1.000000000000000000 ) ) ;
#63488=AXIS2_PLACEMENT_3D ( 'NONE', #124083, #103807, #94615 ) ;
#63489=EDGE_CURVE ( 'NONE', #6418, #68683, #81220, .T. ) ;
#63490=CIRCLE ( 'NONE', #11236, 0.1000000000000002554 ) ;
#63491=DIRECTION ( 'NONE',  ( 0.000000000000000000, 1.000000000000000000, 0.000000000000000000 ) ) ;
#63492=DIRECTION ( 'NONE',  ( -0.000000000000000000, 1.000000000000000000, -0.000000000000000000 ) ) ;
#63493=EDGE_CURVE ( 'NONE', #50907, #120378, #90698, .T. ) ;
#63494=DIRECTION ( 'NONE',  ( 0.000000000000000000, 0.000000000000000000, 1.000000000000000000 ) ) ;
#63495=CARTESIAN_POINT ( 'NONE',  ( -12.49999999999999289, 2.500000000000000000, 3.637306695894644726 ) ) ;
#63496=FACE_OUTER_BOUND ( 'NONE', #25700, .T. ) ;
#63498=CARTESIAN_POINT ( 'NONE',  ( -1.450000000000035483, 2.500000000000000000, 1.818653347947321475 ) ) ;
#63499=EDGE_CURVE ( 'NONE', #69394, #95323, #58243, .T. ) ;
#63500=CIRCLE ( 'NONE', #2953, 0.1000000000000002554 ) ;
#63501=AXIS2_PLACEMENT_3D ( 'NONE', #82190, #103112, #120182 ) ;
#63502=DIRECTION ( 'NONE',  ( -0.000000000000000000, -1.000000000000000000, -0.000000000000000000 ) ) ;
#63503=EDGE_CURVE ( 'NONE', #82453, #75790, #28991, .T. ) ;
#63504=AXIS2_PLACEMENT_3D ( 'NONE', #4860, #92615, #43534 ) ;
#63505=EDGE_CURVE ( 'NONE', #119953, #81870, #77173, .T. ) ;
#63506=VERTEX_POINT ( 'NONE', #62542 ) ;
#63507=CIRCLE ( 'NONE', #11250, 0.1000000000000002554 ) ;
#63508=ADVANCED_FACE ( 'NONE', ( #103745 ), #118864, .T. ) ;
#63509=DIRECTION ( 'NONE',  ( 0.000000000000000000, 0.000000000000000000, -1.000000000000000000 ) ) ;
#63510=EDGE_LOOP ( 'NONE', ( #37537, #54489 ) ) ;
#63511=VERTEX_POINT ( 'NONE', #74289 ) ;
#63512=DIRECTION ( 'NONE',  ( 0.000000000000000000, 0.000000000000000000, 1.000000000000000000 ) ) ;
#63513=CARTESIAN_POINT ( 'NONE',  ( 7.099999999999927702, 12.50000000000000000, 5.022947341949748790 ) ) ;
#63514=AXIS2_PLACEMENT_3D ( 'NONE', #30487, #10184, #57999 ) ;
#63515=DIRECTION ( 'NONE',  ( 0.000000000000000000, 1.000000000000000000, 0.000000000000000000 ) ) ;
#63516=ADVANCED_FACE ( 'NONE', ( #22625 ), #123375, .T. ) ;
#63517=DIRECTION ( 'NONE',  ( 0.000000000000000000, 1.000000000000000000, 0.000000000000000000 ) ) ;
#63518=LINE ( 'NONE', #33423, #115465 ) ;
#63519=VECTOR ( 'NONE', #117300, 1000.000000000000000 ) ;
#63521=AXIS2_PLACEMENT_3D ( 'NONE', #67148, #67820, #6941 ) ;
#63522=DIRECTION ( 'NONE',  ( 0.000000000000000000, 1.000000000000000000, 0.000000000000000000 ) ) ;
#63523=VERTEX_POINT ( 'NONE', #12759 ) ;
#63524=DIRECTION ( 'NONE',  ( -0.000000000000000000, 1.000000000000000000, -0.000000000000000000 ) ) ;
#63525=AXIS2_PLACEMENT_3D ( 'NONE', #55849, #65667, #123307 ) ;
#63526=CARTESIAN_POINT ( 'NONE',  ( 2.899999999999946620, 12.50000000000000000, 0.7579135962115869374 ) ) ;
#63527=VERTEX_POINT ( 'NONE', #23235 ) ;
#63528=ORIENTED_EDGE ( 'NONE', *, *, #41317, .F. ) ;
#63529=EDGE_LOOP ( 'NONE', ( #29816, #15302, #118723, #20104 ) ) ;
#63530=ADVANCED_FACE ( 'NONE', ( #102456 ), #100000, .T. ) ;
#63531=ORIENTED_EDGE ( 'NONE', *, *, #65735, .T. ) ;
#63532=CARTESIAN_POINT ( 'NONE',  ( -9.150000000000009237, 2.500000000000000000, 1.572243186433545548 ) ) ;
#63533=CARTESIAN_POINT ( 'NONE',  ( -0.8500000000000390576, 2.500000000000000000, -6.395190528383301931 ) ) ;
#63534=DIRECTION ( 'NONE',  ( 0.000000000000000000, -0.9999939076577903929, 0.003490651415223739937 ) ) ;
#63535=DIRECTION ( 'NONE',  ( 0.000000000000000000, 1.000000000000000000, 0.000000000000000000 ) ) ;
#63536=FACE_OUTER_BOUND ( 'NONE', #84190, .T. ) ;
#63537=VERTEX_POINT ( 'NONE', #54624 ) ;
#63538=DIRECTION ( 'NONE',  ( 0.000000000000000000, 1.000000000000000000, 0.000000000000000000 ) ) ;
#63539=CARTESIAN_POINT ( 'NONE',  ( -11.25000000000000000, 2.500000000000000000, 7.088010851410848190 ) ) ;
#63540=FACE_OUTER_BOUND ( 'NONE', #43471, .T. ) ;
#63541=DIRECTION ( 'NONE',  ( 0.000000000000000000, 0.000000000000000000, -1.000000000000000000 ) ) ;
#63542=EDGE_LOOP ( 'NONE', ( #65839, #63247 ) ) ;
#63544=CIRCLE ( 'NONE', #23835, 0.06509327318403745899 ) ;
#63545=EDGE_CURVE ( 'NONE', #110508, #47163, #43582, .T. ) ;
#63546=AXIS2_PLACEMENT_3D ( 'NONE', #48092, #56594, #49395 ) ;
#63547=ORIENTED_EDGE ( 'NONE', *, *, #122850, .T. ) ;
#63548=AXIS2_PLACEMENT_3D ( 'NONE', #63157, #72354, #103085 ) ;
#63550=CIRCLE ( 'NONE', #6785, 0.06509327318403745899 ) ;
#63551=CARTESIAN_POINT ( 'NONE',  ( 0.6499999999999543920, 2.500000000000000000, 6.248780366869521430 ) ) ;
#63552=PLANE ( 'NONE',  #71821 ) ;
#63553=CARTESIAN_POINT ( 'NONE',  ( 8.149999999999920419, 2.500000000000000000, 6.941600689897073018 ) ) ;
#63554=AXIS2_PLACEMENT_3D ( 'NONE', #68044, #7830, #47776 ) ;
#63555=AXIS2_PLACEMENT_3D ( 'NONE', #44503, #45806, #15014 ) ;
#63556=CONICAL_SURFACE ( 'NONE', #23846, 0.1000000000000002554, 0.003490658503988666988 ) ;
#63557=CONICAL_SURFACE ( 'NONE', #84383, 0.09999999999999982514, 0.003490658503988666988 ) ;
#63558=ORIENTED_EDGE ( 'NONE', *, *, #128478, .F. ) ;
#63559=DIRECTION ( 'NONE',  ( -0.000000000000000000, 1.000000000000000000, -0.000000000000000000 ) ) ;
#63560=CARTESIAN_POINT ( 'NONE',  ( -9.150000000000011013, 2.500000000000000000, -5.802370205355744659 ) ) ;
#63561=EDGE_CURVE ( 'NONE', #94318, #116685, #93737, .T. ) ;
#63562=CARTESIAN_POINT ( 'NONE',  ( -1.250000000000037526, 2.500000000000000000, -5.902370205355750521 ) ) ;
#63563=CARTESIAN_POINT ( 'NONE',  ( -11.64999999999999680, 2.500000000000000000, 5.802370205355744659 ) ) ;
#63564=CARTESIAN_POINT ( 'NONE',  ( -5.450000000000023270, 2.500000000000000000, -2.165063509461101710 ) ) ;
#63565=VECTOR ( 'NONE', #10040, 1000.000000000000000 ) ;
#63566=EDGE_LOOP ( 'NONE', ( #29372, #17742 ) ) ;
#63568=EDGE_LOOP ( 'NONE', ( #73836, #56122 ) ) ;
#63569=DIRECTION ( 'NONE',  ( 0.000000000000000000, 0.000000000000000000, 1.000000000000000000 ) ) ;
#63570=DIRECTION ( 'NONE',  ( 0.000000000000000000, 0.000000000000000000, 1.000000000000000000 ) ) ;
#63571=CARTESIAN_POINT ( 'NONE',  ( 7.299999999999926104, 2.500000000000000000, -3.983716857408426293 ) ) ;
#63572=CIRCLE ( 'NONE', #59389, 0.06509327318403745899 ) ;
#63574=PLANE ( 'NONE',  #12254 ) ;
#63575=VERTEX_POINT ( 'NONE', #4874 ) ;
#63576=ORIENTED_EDGE ( 'NONE', *, *, #99081, .T. ) ;
#63577=DIRECTION ( 'NONE',  ( -0.000000000000000000, -1.000000000000000000, -0.000000000000000000 ) ) ;
#63578=CARTESIAN_POINT ( 'NONE',  ( -5.400000000000020783, 12.50000000000000000, 5.022947341949748790 ) ) ;
#63579=CARTESIAN_POINT ( 'NONE',  ( -9.200000000000006395, 2.500000000000000000, -0.1000000000000023925 ) ) ;
#63580=DIRECTION ( 'NONE',  ( 0.000000000000000000, 1.000000000000000000, 0.000000000000000000 ) ) ;
#63581=ORIENTED_EDGE ( 'NONE', *, *, #87112, .T. ) ;
#63582=CIRCLE ( 'NONE', #13393, 0.1000000000000002554 ) ;
#63583=AXIS2_PLACEMENT_3D ( 'NONE', #12527, #63580, #23010 ) ;
#63584=DIRECTION ( 'NONE',  ( 0.000000000000000000, 0.000000000000000000, -1.000000000000000000 ) ) ;
#63585=ADVANCED_FACE ( 'NONE', ( #34375 ), #35257, .T. ) ;
#63586=CARTESIAN_POINT ( 'NONE',  ( -1.900000000000035438, 2.500000000000000000, 3.883716857408420431 ) ) ;
#63587=VERTEX_POINT ( 'NONE', #82827 ) ;
#63588=CARTESIAN_POINT ( 'NONE',  ( -5.850000000000018296, 12.50000000000000000, 1.472243186433545459 ) ) ;
#63589=ORIENTED_EDGE ( 'NONE', *, *, #7139, .T. ) ;
#63590=EDGE_CURVE ( 'NONE', #46426, #85762, #97930, .T. ) ;
#63591=DIRECTION ( 'NONE',  ( -0.000000000000000000, -1.000000000000000000, -0.000000000000000000 ) ) ;
#63592=ORIENTED_EDGE ( 'NONE', *, *, #36383, .F. ) ;
#63593=DIRECTION ( 'NONE',  ( 0.000000000000000000, 0.000000000000000000, 1.000000000000000000 ) ) ;
#63594=FACE_OUTER_BOUND ( 'NONE', #45689, .T. ) ;
#63595=EDGE_CURVE ( 'NONE', #73050, #14821, #83474, .T. ) ;
#63596=EDGE_LOOP ( 'NONE', ( #98346, #78475 ) ) ;
#63597=EDGE_CURVE ( 'NONE', #80507, #3939, #2298, .T. ) ;
#63598=EDGE_LOOP ( 'NONE', ( #94255, #42559 ) ) ;
#63599=ADVANCED_FACE ( 'NONE', ( #82170 ), #39573, .T. ) ;
#63600=EDGE_CURVE ( 'NONE', #65132, #89806, #54001, .T. ) ;
#63602=CARTESIAN_POINT ( 'NONE',  ( 10.64999999999990976, 2.500000000000000000, -6.841600689897077814 ) ) ;
#63605=CARTESIAN_POINT ( 'NONE',  ( -2.700000000000029932, 12.50000000000000000, -0.3464101615137782364 ) ) ;
#63606=CARTESIAN_POINT ( 'NONE',  ( 1.649999999999951061, 2.500000000000000000, -6.395190528383301931 ) ) ;
#63608=CIRCLE ( 'NONE', #30264, 0.09999999999999982514 ) ;
#63609=DIRECTION ( 'NONE',  ( 0.000000000000000000, 1.000000000000000000, 0.000000000000000000 ) ) ;
#63611=CIRCLE ( 'NONE', #21754, 0.06509327318403745899 ) ;
#63612=EDGE_CURVE ( 'NONE', #47637, #107914, #3932, .T. ) ;
#63613=ADVANCED_FACE ( 'NONE', ( #42250 ), #75045, .T. ) ;
#63614=ORIENTED_EDGE ( 'NONE', *, *, #92577, .F. ) ;
#63615=EDGE_LOOP ( 'NONE', ( #113085, #32794, #82546, #53292 ) ) ;
#63616=DIRECTION ( 'NONE',  ( -0.000000000000000000, -1.000000000000000000, -0.000000000000000000 ) ) ;
#63617=VERTEX_POINT ( 'NONE', #4231 ) ;
#63618=FACE_OUTER_BOUND ( 'NONE', #28430, .T. ) ;
#63619=CARTESIAN_POINT ( 'NONE',  ( -9.600000000000006750, 2.500000000000000000, 3.537306695894645081 ) ) ;
#63620=DIRECTION ( 'NONE',  ( 0.000000000000000000, 0.000000000000000000, 1.000000000000000000 ) ) ;
#63621=ORIENTED_EDGE ( 'NONE', *, *, #92037, .T. ) ;
#63622=ORIENTED_EDGE ( 'NONE', *, *, #127421, .F. ) ;
#63623=CARTESIAN_POINT ( 'NONE',  ( 0.7999999999999548583, 12.50000000000000000, 4.395220292106234439 ) ) ;
#63624=VERTEX_POINT ( 'NONE', #104384 ) ;
#63625=DIRECTION ( 'NONE',  ( 0.000000000000000000, 0.000000000000000000, 1.000000000000000000 ) ) ;
#63626=CARTESIAN_POINT ( 'NONE',  ( -12.49999999999995737, 12.50000000000000000, 4.395220292106234439 ) ) ;
#63627=DIRECTION ( 'NONE',  ( -0.000000000000000000, 1.000000000000000000, -0.000000000000000000 ) ) ;
#63628=DIRECTION ( 'NONE',  ( 0.000000000000000000, 0.000000000000000000, 1.000000000000000000 ) ) ;
#63629=DIRECTION ( 'NONE',  ( -4.274815082592931898E-19, -0.9999939076577903929, -0.003490651415223739937 ) ) ;
#63630=AXIS2_PLACEMENT_3D ( 'NONE', #80582, #41312, #41952 ) ;
#63631=DIRECTION ( 'NONE',  ( 0.000000000000000000, 0.000000000000000000, 1.000000000000000000 ) ) ;
#63632=CIRCLE ( 'NONE', #2987, 0.09999999999999982514 ) ;
#63633=DIRECTION ( 'NONE',  ( 0.000000000000000000, 0.000000000000000000, -1.000000000000000000 ) ) ;
#63634=DIRECTION ( 'NONE',  ( -4.274815082592931898E-19, -0.9999939076577903929, -0.003490651415223739937 ) ) ;
#63635=AXIS2_PLACEMENT_3D ( 'NONE', #3103, #41106, #102568 ) ;
#63637=CARTESIAN_POINT ( 'NONE',  ( -3.750000000000027534, 2.500000000000000000, 2.857883832488649301 ) ) ;
#63638=CARTESIAN_POINT ( 'NONE',  ( -3.749999999999991118, 2.500000000000000000, -2.265063509461101798 ) ) ;
#63639=VECTOR ( 'NONE', #32690, 1000.000000000000000 ) ;
#63640=VECTOR ( 'NONE', #119038, 1000.000000000000000 ) ;
#63641=EDGE_LOOP ( 'NONE', ( #52669, #50260 ) ) ;
#63642=VERTEX_POINT ( 'NONE', #14688 ) ;
#63643=VERTEX_POINT ( 'NONE', #94551 ) ;
#63644=AXIS2_PLACEMENT_3D ( 'NONE', #40873, #110855, #31670 ) ;
#63646=ORIENTED_EDGE ( 'NONE', *, *, #124067, .T. ) ;
#63647=LINE ( 'NONE', #26131, #61225 ) ;
#63649=VERTEX_POINT ( 'NONE', #86670 ) ;
#63650=ORIENTED_EDGE ( 'NONE', *, *, #48656, .T. ) ;
#63651=CARTESIAN_POINT ( 'NONE',  ( 10.64999999999991331, 12.50000000000000000, -1.818653347947325916 ) ) ;
#63652=AXIS2_PLACEMENT_3D ( 'NONE', #38581, #9090, #106646 ) ;
#63653=AXIS2_PLACEMENT_3D ( 'NONE', #94187, #74548, #124300 ) ;
#63654=CARTESIAN_POINT ( 'NONE',  ( -8.550000000000014921, 12.50000000000000000, -6.148780366869520897 ) ) ;
#63655=( NAMED_UNIT ( * ) SI_UNIT ( $, .STERADIAN. ) SOLID_ANGLE_UNIT ( ) );
#63656=DIRECTION ( 'NONE',  ( 0.000000000000000000, 0.000000000000000000, 1.000000000000000000 ) ) ;
#63657=DIRECTION ( 'NONE',  ( 0.000000000000000000, 0.000000000000000000, 1.000000000000000000 ) ) ;
#63658=CONICAL_SURFACE ( 'NONE', #105409, 0.1000000000000002554, 0.003490658503988666988 ) ;
#63660=ORIENTED_EDGE ( 'NONE', *, *, #36315, .T. ) ;
#63661=ADVANCED_FACE ( 'NONE', ( #127261 ), #106316, .T. ) ;
#63662=CARTESIAN_POINT ( 'NONE',  ( -3.300000000000028244, 12.50000000000000000, 4.395220292106234439 ) ) ;
#63663=ORIENTED_EDGE ( 'NONE', *, *, #47233, .F. ) ;
#63664=ADVANCED_FACE ( 'NONE', ( #55921 ), #41616, .T. ) ;
#63665=EDGE_LOOP ( 'NONE', ( #83762, #103866, #103219, #70425 ) ) ;
#63666=ORIENTED_EDGE ( 'NONE', *, *, #56749, .F. ) ;
#63667=ADVANCED_FACE ( 'NONE', ( #35649 ), #15982, .T. ) ;
#63668=DIRECTION ( 'NONE',  ( 0.000000000000000000, 0.000000000000000000, -1.000000000000000000 ) ) ;
#63669=EDGE_LOOP ( 'NONE', ( #110012, #81514, #123190, #128090 ) ) ;
#63670=VERTEX_POINT ( 'NONE', #77496 ) ;
#63671=ORIENTED_EDGE ( 'NONE', *, *, #12360, .F. ) ;
#63672=CIRCLE ( 'NONE', #82544, 0.06509327318403745899 ) ;
#63673=DIRECTION ( 'NONE',  ( 0.000000000000000000, 0.000000000000000000, 1.000000000000000000 ) ) ;
#63674=EDGE_CURVE ( 'NONE', #5720, #29188, #5518, .T. ) ;
#63675=LINE ( 'NONE', #64932, #129205 ) ;
#63676=DIRECTION ( 'NONE',  ( -0.000000000000000000, 1.000000000000000000, -0.000000000000000000 ) ) ;
#63677=FACE_OUTER_BOUND ( 'NONE', #13571, .T. ) ;
#63678=DIRECTION ( 'NONE',  ( -0.000000000000000000, 1.000000000000000000, -0.000000000000000000 ) ) ;
#63679=FACE_OUTER_BOUND ( 'NONE', #13403, .T. ) ;
#63680=DIRECTION ( 'NONE',  ( -0.000000000000000000, 1.000000000000000000, -0.000000000000000000 ) ) ;
#63681=AXIS2_PLACEMENT_3D ( 'NONE', #117502, #27871, #40278 ) ;
#63682=CIRCLE ( 'NONE', #49023, 0.09999999999999982514 ) ;
#63683=ORIENTED_EDGE ( 'NONE', *, *, #48625, .F. ) ;
#63684=DIRECTION ( 'NONE',  ( 0.000000000000000000, 1.000000000000000000, 0.000000000000000000 ) ) ;
#63685=ORIENTED_EDGE ( 'NONE', *, *, #98476, .T. ) ;
#63686=LINE ( 'NONE', #85247, #31506 ) ;
#63688=EDGE_CURVE ( 'NONE', #48618, #16035, #72898, .T. ) ;
#63689=ORIENTED_EDGE ( 'NONE', *, *, #68310, .F. ) ;
#63690=LINE ( 'NONE', #74148, #59488 ) ;
#63692=CONICAL_SURFACE ( 'NONE', #65811, 0.1000000000000002554, 0.003490658503988666988 ) ;
#63693=DIRECTION ( 'NONE',  ( -0.000000000000000000, -1.000000000000000000, -0.000000000000000000 ) ) ;
#63694=AXIS2_PLACEMENT_3D ( 'NONE', #125091, #24957, #74059 ) ;
#63695=VERTEX_POINT ( 'NONE', #125312 ) ;
#63696=VERTEX_POINT ( 'NONE', #16626 ) ;
#63697=CARTESIAN_POINT ( 'NONE',  ( -4.150000000000025224, 2.500000000000000000, 2.957883832488649389 ) ) ;
#63698=DIRECTION ( 'NONE',  ( -0.000000000000000000, 1.000000000000000000, -0.000000000000000000 ) ) ;
#63699=DIRECTION ( 'NONE',  ( 0.000000000000000000, 0.000000000000000000, -1.000000000000000000 ) ) ;
#63701=DIRECTION ( 'NONE',  ( -0.000000000000000000, -1.000000000000000000, -0.000000000000000000 ) ) ;
#63702=ORIENTED_EDGE ( 'NONE', *, *, #44074, .T. ) ;
#63703=CONICAL_SURFACE ( 'NONE', #42977, 0.09999999999999982514, 0.003490658503988666988 ) ;
#63704=AXIS2_PLACEMENT_3D ( 'NONE', #107719, #129321, #127367 ) ;
#63705=ADVANCED_FACE ( 'NONE', ( #67015 ), #64568, .T. ) ;
#63706=EDGE_LOOP ( 'NONE', ( #49988, #44882, #90705, #70191 ) ) ;
#63707=CIRCLE ( 'NONE', #7237, 0.06509327318403745899 ) ;
#63708=FACE_OUTER_BOUND ( 'NONE', #98281, .T. ) ;
#63709=CARTESIAN_POINT ( 'NONE',  ( 8.349999999999919709, 12.50000000000000000, 5.802370205355744659 ) ) ;
#63711=DIRECTION ( 'NONE',  ( -0.000000000000000000, 1.000000000000000000, -0.000000000000000000 ) ) ;
#63712=DIRECTION ( 'NONE',  ( 0.000000000000000000, 1.000000000000000000, 0.000000000000000000 ) ) ;
#63713=EDGE_CURVE ( 'NONE', #105557, #55712, #87942, .T. ) ;
#63714=DIRECTION ( 'NONE',  ( -4.274815082592931898E-19, -0.9999939076577903929, -0.003490651415223739937 ) ) ;
#63715=DIRECTION ( 'NONE',  ( 0.000000000000000000, 1.000000000000000000, 0.000000000000000000 ) ) ;
#63716=ORIENTED_EDGE ( 'NONE', *, *, #39384, .F. ) ;
#63717=DIRECTION ( 'NONE',  ( 0.000000000000000000, -0.000000000000000000, 1.000000000000000000 ) ) ;
#63718=AXIS2_PLACEMENT_3D ( 'NONE', #128248, #45813, #38586 ) ;
#63719=CARTESIAN_POINT ( 'NONE',  ( 13.54999999999989591, 2.500000000000000000, -1.818653347947326138 ) ) ;
#63720=CARTESIAN_POINT ( 'NONE',  ( 9.199999999999919353, 2.500000000000000000, -0.1000000000000022815 ) ) ;
#63721=VECTOR ( 'NONE', #61927, 1000.000000000000000 ) ;
#63722=EDGE_LOOP ( 'NONE', ( #48982, #64708, #58781, #55863 ) ) ;
#63723=CIRCLE ( 'NONE', #57462, 0.06509327318403745899 ) ;
#63725=EDGE_CURVE ( 'NONE', #29090, #74701, #115461, .T. ) ;
#63726=DIRECTION ( 'NONE',  ( 0.000000000000000000, 1.000000000000000000, 0.000000000000000000 ) ) ;
#63727=CIRCLE ( 'NONE', #24015, 0.1000000000000002554 ) ;
#63728=AXIS2_PLACEMENT_3D ( 'NONE', #6434, #88223, #128190 ) ;
#63729=ORIENTED_EDGE ( 'NONE', *, *, #113743, .F. ) ;
#63730=LINE ( 'NONE', #122645, #27938 ) ;
#63731=AXIS2_PLACEMENT_3D ( 'NONE', #30565, #29264, #71105 ) ;
#63732=EDGE_LOOP ( 'NONE', ( #92197, #84860 ) ) ;
#63733=FACE_OUTER_BOUND ( 'NONE', #122580, .T. ) ;
#63734=DIRECTION ( 'NONE',  ( 0.000000000000000000, 0.000000000000000000, 1.000000000000000000 ) ) ;
#63735=DIRECTION ( 'NONE',  ( 0.000000000000000000, 0.000000000000000000, 1.000000000000000000 ) ) ;
#63736=EDGE_LOOP ( 'NONE', ( #9969, #22915, #16956, #4223 ) ) ;
#63737=AXIS2_PLACEMENT_3D ( 'NONE', #57400, #97958, #58688 ) ;
#63738=CIRCLE ( 'NONE', #118101, 0.1000000000000000472 ) ;
#63739=CARTESIAN_POINT ( 'NONE',  ( -11.24999999999996270, 2.500000000000000000, 6.595190528383296780 ) ) ;
#63740=EDGE_CURVE ( 'NONE', #104745, #32777, #45807, .T. ) ;
#63741=CARTESIAN_POINT ( 'NONE',  ( -3.350000000000028955, 12.50000000000000000, 5.737276932171707422 ) ) ;
#63742=ORIENTED_EDGE ( 'NONE', *, *, #41288, .T. ) ;
#63743=EDGE_CURVE ( 'NONE', #114031, #10654, #36942, .T. ) ;
#63744=ORIENTED_EDGE ( 'NONE', *, *, #65790, .F. ) ;
#63746=DIRECTION ( 'NONE',  ( 0.000000000000000000, 1.000000000000000000, 0.000000000000000000 ) ) ;
#63747=DIRECTION ( 'NONE',  ( 0.000000000000000000, 1.000000000000000000, 0.000000000000000000 ) ) ;
#63748=DIRECTION ( 'NONE',  ( 0.000000000000000000, 0.000000000000000000, 1.000000000000000000 ) ) ;
#63749=EDGE_CURVE ( 'NONE', #86969, #46288, #35342, .T. ) ;
#63750=EDGE_CURVE ( 'NONE', #29271, #108499, #22833, .T. ) ;
#63751=VERTEX_POINT ( 'NONE', #86007 ) ;
#63752=EDGE_CURVE ( 'NONE', #26581, #105656, #118063, .T. ) ;
#63753=EDGE_CURVE ( 'NONE', #12555, #71950, #121011, .T. ) ;
#63754=DIRECTION ( 'NONE',  ( 0.000000000000000000, 1.000000000000000000, 0.000000000000000000 ) ) ;
#63755=CARTESIAN_POINT ( 'NONE',  ( 0.4499999999999569344, 12.50000000000000000, 2.165063509461097713 ) ) ;
#63756=AXIS2_PLACEMENT_3D ( 'NONE', #128517, #60411, #29008 ) ;
#63757=ORIENTED_EDGE ( 'NONE', *, *, #55823, .F. ) ;
#63758=DIRECTION ( 'NONE',  ( 0.000000000000000000, 0.000000000000000000, 1.000000000000000000 ) ) ;
#63759=DIRECTION ( 'NONE',  ( 0.000000000000000000, 0.000000000000000000, 1.000000000000000000 ) ) ;
#63760=ADVANCED_FACE ( 'NONE', ( #28411 ), #112701, .T. ) ;
#63762=PLANE ( 'NONE',  #126552 ) ;
#63764=EDGE_CURVE ( 'NONE', #59178, #79801, #93825, .T. ) ;
#63765=CARTESIAN_POINT ( 'NONE',  ( -9.800000000000004263, 12.50000000000000000, -0.3464101615137783474 ) ) ;
#63766=CARTESIAN_POINT ( 'NONE',  ( 6.449999999999931788, 2.500000000000000000, -6.148780366869526226 ) ) ;
#63767=CONICAL_SURFACE ( 'NONE', #7309, 0.09999999999999982514, 0.003490658503988666988 ) ;
#63768=CIRCLE ( 'NONE', #80503, 0.06509327318403745899 ) ;
#63769=ADVANCED_FACE ( 'NONE', ( #95217 ), #79262, .T. ) ;
#63770=EDGE_CURVE ( 'NONE', #90867, #35444, #33205, .T. ) ;
#63771=ORIENTED_EDGE ( 'NONE', *, *, #59204, .T. ) ;
#63772=ORIENTED_EDGE ( 'NONE', *, *, #98139, .T. ) ;
#63774=ORIENTED_EDGE ( 'NONE', *, *, #3194, .T. ) ;
#63775=DIRECTION ( 'NONE',  ( -0.000000000000000000, -1.000000000000000000, -0.000000000000000000 ) ) ;
#63776=DIRECTION ( 'NONE',  ( 0.000000000000000000, 1.000000000000000000, 0.000000000000000000 ) ) ;
#63777=DIRECTION ( 'NONE',  ( 0.000000000000000000, 0.000000000000000000, -1.000000000000000000 ) ) ;
#63778=EDGE_LOOP ( 'NONE', ( #63316, #15753, #75519, #89314 ) ) ;
#63779=FACE_BOUND ( 'NONE', #8542, .T. ) ;
#63780=ADVANCED_FACE ( 'NONE', ( #29066 ), #112613, .T. ) ;
#63781=CARTESIAN_POINT ( 'NONE',  ( 3.349999999999944578, 2.500000000000000000, -1.472243186433550122 ) ) ;
#63782=DIRECTION ( 'NONE',  ( 0.000000000000000000, 0.000000000000000000, 1.000000000000000000 ) ) ;
#63783=AXIS2_PLACEMENT_3D ( 'NONE', #43936, #4605, #32832 ) ;
#63784=DIRECTION ( 'NONE',  ( 0.000000000000000000, 1.000000000000000000, 0.000000000000000000 ) ) ;
#63785=DIRECTION ( 'NONE',  ( 0.000000000000000000, 0.000000000000000000, 1.000000000000000000 ) ) ;
#63786=AXIS2_PLACEMENT_3D ( 'NONE', #81777, #11101, #111229 ) ;
#63787=CARTESIAN_POINT ( 'NONE',  ( -14.99999999999998224, 12.50000000000000000, -0.6277270498435144619 ) ) ;
#63788=DIRECTION ( 'NONE',  ( 0.000000000000000000, 0.000000000000000000, 1.000000000000000000 ) ) ;
#63789=DIRECTION ( 'NONE',  ( -0.000000000000000000, 1.000000000000000000, -0.000000000000000000 ) ) ;
#63790=PLANE ( 'NONE',  #67951 ) ;
#63791=DIRECTION ( 'NONE',  ( 0.000000000000000000, 1.000000000000000000, 0.000000000000000000 ) ) ;
#63792=CARTESIAN_POINT ( 'NONE',  ( 3.749999999999942268, 12.50000000000000000, -1.472243186433550122 ) ) ;
#63793=VERTEX_POINT ( 'NONE', #51291 ) ;
#63795=ORIENTED_EDGE ( 'NONE', *, *, #59740, .F. ) ;
#63796=EDGE_LOOP ( 'NONE', ( #116608, #61822, #22958, #89430 ) ) ;
#63797=VECTOR ( 'NONE', #84699, 1000.000000000000000 ) ;
#63798=VERTEX_POINT ( 'NONE', #70913 ) ;
#63799=ORIENTED_EDGE ( 'NONE', *, *, #90027, .F. ) ;
#63800=ORIENTED_EDGE ( 'NONE', *, *, #101920, .F. ) ;
#63801=FACE_OUTER_BOUND ( 'NONE', #114070, .T. ) ;
#63802=ORIENTED_EDGE ( 'NONE', *, *, #32597, .F. ) ;
#63803=ORIENTED_EDGE ( 'NONE', *, *, #27193, .F. ) ;
#63804=CARTESIAN_POINT ( 'NONE',  ( 14.37945523737784725, -2.500000000000446310, 7.667852709071338424 ) ) ;
#63805=DIRECTION ( 'NONE',  ( 0.000000000000000000, 0.000000000000000000, 1.000000000000000000 ) ) ;
#63806=DIRECTION ( 'NONE',  ( -0.000000000000000000, 1.000000000000000000, -0.000000000000000000 ) ) ;
#63807=EDGE_LOOP ( 'NONE', ( #42413, #102764, #117228, #5256 ) ) ;
#63808=CARTESIAN_POINT ( 'NONE',  ( 6.649999999999930189, 2.500000000000000000, 5.902370205355745192 ) ) ;
#63809=ORIENTED_EDGE ( 'NONE', *, *, #72932, .F. ) ;
#63810=EDGE_CURVE ( 'NONE', #49718, #128241, #108485, .T. ) ;
#63811=AXIS2_PLACEMENT_3D ( 'NONE', #19321, #100474, #99847 ) ;
#63812=ORIENTED_EDGE ( 'NONE', *, *, #27743, .F. ) ;
#63813=CARTESIAN_POINT ( 'NONE',  ( 1.049999999999952083, 2.500000000000000000, 6.741600689897071952 ) ) ;
#63814=ORIENTED_EDGE ( 'NONE', *, *, #59792, .T. ) ;
#63816=ADVANCED_FACE ( 'NONE', ( #71542 ), #21153, .T. ) ;
#63817=VECTOR ( 'NONE', #117871, 1000.000000000000000 ) ;
#63819=ORIENTED_EDGE ( 'NONE', *, *, #84207, .T. ) ;
#63821=DIRECTION ( 'NONE',  ( 0.000000000000000000, 0.000000000000000000, 1.000000000000000000 ) ) ;
#63822=CONICAL_SURFACE ( 'NONE', #111939, 0.09999999999999999167, 0.003490658503988666988 ) ;
#63823=CARTESIAN_POINT ( 'NONE',  ( -10.40000000000000213, 12.50000000000000000, -4.957854068765712441 ) ) ;
#63824=DIRECTION ( 'NONE',  ( -4.274815082592931898E-19, -0.9999939076577903929, -0.003490651415223739937 ) ) ;
#63825=DIRECTION ( 'NONE',  ( -0.000000000000000000, -1.000000000000000000, -0.000000000000000000 ) ) ;
#63826=CIRCLE ( 'NONE', #53363, 0.06509327318403745899 ) ;
#63827=DIRECTION ( 'NONE',  ( 0.000000000000000000, 1.000000000000000000, 0.000000000000000000 ) ) ;
#63828=ORIENTED_EDGE ( 'NONE', *, *, #10364, .F. ) ;
#63829=CARTESIAN_POINT ( 'NONE',  ( 7.899999999999924860, 12.50000000000000000, 3.572213422710607489 ) ) ;
#63830=AXIS2_PLACEMENT_3D ( 'NONE', #84773, #54026, #125342 ) ;
#63831=CIRCLE ( 'NONE', #74296, 0.06509327318403745899 ) ;
#63832=VERTEX_POINT ( 'NONE', #88612 ) ;
#63833=CARTESIAN_POINT ( 'NONE',  ( 17.50000000000000000, 2.499999999999999556, -0.6666666666666630769 ) ) ;
#63834=ORIENTED_EDGE ( 'NONE', *, *, #52357, .F. ) ;
#63835=DIRECTION ( 'NONE',  ( -0.000000000000000000, -1.000000000000000000, -0.000000000000000000 ) ) ;
#63836=DIRECTION ( 'NONE',  ( 0.000000000000000000, 0.000000000000000000, 1.000000000000000000 ) ) ;
#63837=VECTOR ( 'NONE', #111668, 1000.000000000000000 ) ;
#63838=LINE ( 'NONE', #42933, #17322 ) ;
#63839=DIRECTION ( 'NONE',  ( 0.000000000000000000, -0.000000000000000000, 1.000000000000000000 ) ) ;
#63840=ORIENTED_EDGE ( 'NONE', *, *, #123193, .T. ) ;
#63841=CARTESIAN_POINT ( 'NONE',  ( 4.549999999999939426, 12.50000000000000000, -2.165063509461101710 ) ) ;
#63842=DIRECTION ( 'NONE',  ( 0.000000000000000000, 1.000000000000000000, 0.000000000000000000 ) ) ;
#63843=ORIENTED_EDGE ( 'NONE', *, *, #113836, .T. ) ;
#63844=EDGE_LOOP ( 'NONE', ( #118292, #117456 ) ) ;
#63845=EDGE_LOOP ( 'NONE', ( #108497, #82698 ) ) ;
#63846=CARTESIAN_POINT ( 'NONE',  ( 0.1999999999999636513, 2.500000000000000000, -0.3464101615137760715 ) ) ;
#63847=CARTESIAN_POINT ( 'NONE',  ( -8.750000000000012434, 2.500000000000000000, -5.702370205355745014 ) ) ;
#63849=AXIS2_PLACEMENT_3D ( 'NONE', #121882, #94346, #113345 ) ;
#63851=EDGE_CURVE ( 'NONE', #10073, #115594, #123075, .T. ) ;
#63853=CARTESIAN_POINT ( 'NONE',  ( -3.750000000000027534, 2.500000000000000000, 2.857883832488649301 ) ) ;
#63854=AXIS2_PLACEMENT_3D ( 'NONE', #91788, #22425, #10620 ) ;
#63855=CIRCLE ( 'NONE', #97302, 0.06509327318403745899 ) ;
#63856=ORIENTED_EDGE ( 'NONE', *, *, #72630, .T. ) ;
#63857=DIRECTION ( 'NONE',  ( 0.000000000000000000, 0.000000000000000000, 1.000000000000000000 ) ) ;
#63858=ORIENTED_EDGE ( 'NONE', *, *, #16981, .F. ) ;
#63859=CARTESIAN_POINT ( 'NONE',  ( 11.44999999999990870, 12.50000000000000000, -1.753560074763288679 ) ) ;
#63860=EDGE_CURVE ( 'NONE', #94655, #17558, #43669, .T. ) ;
#63861=DIRECTION ( 'NONE',  ( -4.274815082592931898E-19, -0.9999939076577903929, -0.003490651415223739937 ) ) ;
#63863=DIRECTION ( 'NONE',  ( 0.000000000000000000, 0.000000000000000000, -1.000000000000000000 ) ) ;
#63864=DIRECTION ( 'NONE',  ( 0.000000000000000000, 1.000000000000000000, 0.000000000000000000 ) ) ;
#63865=EDGE_LOOP ( 'NONE', ( #44520, #34364, #102899, #73533 ) ) ;
#63866=VECTOR ( 'NONE', #128954, 1000.000000000000000 ) ;
#63867=CONICAL_SURFACE ( 'NONE', #26213, 0.09999999999999999167, 0.003490658503988666988 ) ;
#63868=LINE ( 'NONE', #42299, #40864 ) ;
#63869=DIRECTION ( 'NONE',  ( -0.000000000000000000, 1.000000000000000000, -0.000000000000000000 ) ) ;
#63870=ORIENTED_EDGE ( 'NONE', *, *, #98746, .T. ) ;
#63871=EDGE_CURVE ( 'NONE', #89315, #74379, #12337, .T. ) ;
#63872=ORIENTED_EDGE ( 'NONE', *, *, #862, .T. ) ;
#63873=CARTESIAN_POINT ( 'NONE',  ( 0.8499999999999553468, 12.50000000000000000, 1.472243186433545459 ) ) ;
#63874=CONICAL_SURFACE ( 'NONE', #38870, 0.09999999999999982514, 0.003490658503988666988 ) ;
#63875=AXIS2_PLACEMENT_3D ( 'NONE', #107569, #97738, #127846 ) ;
#63876=ORIENTED_EDGE ( 'NONE', *, *, #12761, .T. ) ;
#63877=ORIENTED_EDGE ( 'NONE', *, *, #107820, .T. ) ;
#63878=CARTESIAN_POINT ( 'NONE',  ( -7.700000000000014388, 12.50000000000000000, -0.3464101615137782364 ) ) ;
#63879=ORIENTED_EDGE ( 'NONE', *, *, #50741, .F. ) ;
#63880=FACE_OUTER_BOUND ( 'NONE', #11202, .T. ) ;
#63881=CARTESIAN_POINT ( 'NONE',  ( 10.84999999999991260, 2.500000000000000000, -1.572243186433550211 ) ) ;
#63883=VERTEX_POINT ( 'NONE', #10668 ) ;
#63884=CONICAL_SURFACE ( 'NONE', #80623, 0.1000000000000002554, 0.003490658503988666988 ) ;
#63885=CARTESIAN_POINT ( 'NONE',  ( -5.000000000000023093, 2.500000000000000000, 0.5928203230275495006 ) ) ;
#63887=ORIENTED_EDGE ( 'NONE', *, *, #84332, .F. ) ;
#63888=CARTESIAN_POINT ( 'NONE',  ( 15.39999999999989200, 2.500000000000000000, 0.5928203230275495006 ) ) ;
#63889=DIRECTION ( 'NONE',  ( -0.000000000000000000, -1.000000000000000000, -0.000000000000000000 ) ) ;
#63890=CONICAL_SURFACE ( 'NONE', #7444, 0.1000000000000000472, 0.003490658503988666988 ) ;
#63891=ORIENTED_EDGE ( 'NONE', *, *, #47225, .F. ) ;
#63892=EDGE_CURVE ( 'NONE', #76783, #100499, #87552, .T. ) ;
#63893=VECTOR ( 'NONE', #55879, 1000.000000000000000 ) ;
#63894=EDGE_LOOP ( 'NONE', ( #60135, #113121 ) ) ;
#63895=AXIS2_PLACEMENT_3D ( 'NONE', #45996, #75430, #115338 ) ;
#63896=EDGE_LOOP ( 'NONE', ( #27377, #121930 ) ) ;
#63897=VERTEX_POINT ( 'NONE', #58527 ) ;
#63898=DIRECTION ( 'NONE',  ( 0.000000000000000000, 0.000000000000000000, 1.000000000000000000 ) ) ;
#63899=CARTESIAN_POINT ( 'NONE',  ( 1.849999999999949019, 2.500000000000000000, 6.941600689897073018 ) ) ;
#63900=CARTESIAN_POINT ( 'NONE',  ( 4.149999999999939959, 2.500000000000000000, 1.472243186433545459 ) ) ;
#63901=ADVANCED_FACE ( 'NONE', ( #121295 ), #66712, .T. ) ;
#63902=FACE_BOUND ( 'NONE', #7514, .T. ) ;
#63903=VERTEX_POINT ( 'NONE', #20527 ) ;
#63905=ADVANCED_FACE ( 'NONE', ( #18584 ), #50002, .T. ) ;
#63906=DIRECTION ( 'NONE',  ( 0.000000000000000000, 0.000000000000000000, 1.000000000000000000 ) ) ;
#63907=CARTESIAN_POINT ( 'NONE',  ( -9.150000000000009237, 2.500000000000000000, -7.188010851410848723 ) ) ;
#63908=AXIS2_PLACEMENT_3D ( 'NONE', #3302, #73975, #32788 ) ;
#63909=ADVANCED_FACE ( 'NONE', ( #90536 ), #116878, .T. ) ;
#63910=DIRECTION ( 'NONE',  ( -0.000000000000000000, 1.000000000000000000, -0.000000000000000000 ) ) ;
#63911=AXIS2_PLACEMENT_3D ( 'NONE', #119394, #70319, #38953 ) ;
#63912=EDGE_CURVE ( 'NONE', #61265, #96534, #125309, .T. ) ;
#63913=LINE ( 'NONE', #33179, #94887 ) ;
#63914=EDGE_CURVE ( 'NONE', #10784, #62494, #119056, .T. ) ;
#63915=CARTESIAN_POINT ( 'NONE',  ( 10.84999999999991260, 12.50000000000000000, -2.922977105672691422 ) ) ;
#63916=CARTESIAN_POINT ( 'NONE',  ( 2.899999999999944844, 2.500000000000000000, 3.537306695894645081 ) ) ;
#63917=AXIS2_PLACEMENT_3D ( 'NONE', #69593, #90519, #30341 ) ;
#63918=EDGE_CURVE ( 'NONE', #64313, #109253, #109548, .T. ) ;
#63919=VERTEX_POINT ( 'NONE', #80740 ) ;
#63920=EDGE_LOOP ( 'NONE', ( #20002, #50133 ) ) ;
#63921=ORIENTED_EDGE ( 'NONE', *, *, #49869, .T. ) ;
#63922=ORIENTED_EDGE ( 'NONE', *, *, #123634, .F. ) ;
#63923=AXIS2_PLACEMENT_3D ( 'NONE', #81244, #2019, #110686 ) ;
#63924=ORIENTED_EDGE ( 'NONE', *, *, #55551, .F. ) ;
#63925=DIRECTION ( 'NONE',  ( 0.000000000000000000, 0.000000000000000000, -1.000000000000000000 ) ) ;
#63926=DIRECTION ( 'NONE',  ( 0.000000000000000000, 0.000000000000000000, 1.000000000000000000 ) ) ;
#63927=ORIENTED_EDGE ( 'NONE', *, *, #24810, .F. ) ;
#63928=FACE_BOUND ( 'NONE', #70082, .T. ) ;
#63929=EDGE_CURVE ( 'NONE', #126052, #47870, #85592, .T. ) ;
#63930=DIRECTION ( 'NONE',  ( -0.000000000000000000, -1.000000000000000000, -0.000000000000000000 ) ) ;
#63931=EDGE_CURVE ( 'NONE', #105257, #38338, #129455, .T. ) ;
#63932=EDGE_LOOP ( 'NONE', ( #36622, #106487, #126181, #83939 ) ) ;
#63933=DIRECTION ( 'NONE',  ( -4.274815082592931898E-19, -0.9999939076577903929, -0.003490651415223739937 ) ) ;
#63934=CARTESIAN_POINT ( 'NONE',  ( 11.24999999999994493, 2.500000000000000000, 6.595190528383296780 ) ) ;
#63935=DIRECTION ( 'NONE',  ( 0.000000000000000000, 0.000000000000000000, 1.000000000000000000 ) ) ;
#63936=AXIS2_PLACEMENT_3D ( 'NONE', #100781, #109983, #100163 ) ;
#63937=EDGE_LOOP ( 'NONE', ( #53945, #122578 ) ) ;
#63938=CARTESIAN_POINT ( 'NONE',  ( 16.56576425164991306, -2.499999999999999556, 6.084390597445977100 ) ) ;
#63939=VERTEX_POINT ( 'NONE', #44674 ) ;
#63940=ORIENTED_EDGE ( 'NONE', *, *, #117058, .F. ) ;
#63941=VERTEX_POINT ( 'NONE', #101665 ) ;
#63942=DIRECTION ( 'NONE',  ( 0.000000000000000000, 0.000000000000000000, 1.000000000000000000 ) ) ;
#63943=DIRECTION ( 'NONE',  ( 0.000000000000000000, 1.000000000000000000, 0.000000000000000000 ) ) ;
#63944=CIRCLE ( 'NONE', #17963, 0.06509327318403743123 ) ;
#63945=CARTESIAN_POINT ( 'NONE',  ( 13.54999999999990123, 2.500000000000000000, 1.818653347947321475 ) ) ;
#63946=ORIENTED_EDGE ( 'NONE', *, *, #74813, .T. ) ;
#63947=CARTESIAN_POINT ( 'NONE',  ( 9.149999999999920419, 12.50000000000000000, 1.537336459617582918 ) ) ;
#63948=AXIS2_PLACEMENT_3D ( 'NONE', #124612, #106881, #57153 ) ;
#63949=AXIS2_PLACEMENT_3D ( 'NONE', #80831, #121381, #91930 ) ;
#63950=FACE_OUTER_BOUND ( 'NONE', #107362, .T. ) ;
#63951=DIRECTION ( 'NONE',  ( 0.000000000000000000, 0.000000000000000000, 1.000000000000000000 ) ) ;
#63953=EDGE_LOOP ( 'NONE', ( #128293, #71240 ) ) ;
#63954=DIRECTION ( 'NONE',  ( 0.000000000000000000, 0.000000000000000000, 1.000000000000000000 ) ) ;
#63955=VERTEX_POINT ( 'NONE', #2806 ) ;
#63956=DIRECTION ( 'NONE',  ( 0.000000000000000000, 0.000000000000000000, 1.000000000000000000 ) ) ;
#63957=CIRCLE ( 'NONE', #28368, 0.1000000000000002554 ) ;
#63958=ORIENTED_EDGE ( 'NONE', *, *, #5515, .F. ) ;
#63959=ADVANCED_FACE ( 'NONE', ( #82008 ), #4088, .T. ) ;
#63960=CIRCLE ( 'NONE', #5447, 0.06509327318403745899 ) ;
#63961=ORIENTED_EDGE ( 'NONE', *, *, #72074, .T. ) ;
#63962=LINE ( 'NONE', #14193, #86860 ) ;
#63963=DIRECTION ( 'NONE',  ( 0.000000000000000000, 1.000000000000000000, 0.000000000000000000 ) ) ;
#63964=CARTESIAN_POINT ( 'NONE',  ( 6.649999999999929301, 2.500000000000000000, -2.265063509461101798 ) ) ;
#63965=DIRECTION ( 'NONE',  ( 0.000000000000000000, -0.000000000000000000, 1.000000000000000000 ) ) ;
#63966=DIRECTION ( 'NONE',  ( 0.000000000000000000, 1.000000000000000000, 0.000000000000000000 ) ) ;
#63967=VERTEX_POINT ( 'NONE', #114058 ) ;
#63968=ORIENTED_EDGE ( 'NONE', *, *, #85722, .T. ) ;
#63969=ADVANCED_FACE ( 'NONE', ( #13256 ), #127372, .T. ) ;
#63970=CARTESIAN_POINT ( 'NONE',  ( 11.64999999999990798, 2.500000000000000000, -2.857883832488653741 ) ) ;
#63971=CONICAL_SURFACE ( 'NONE', #115903, 0.1000000000000000056, 0.003490658503988666988 ) ;
#63972=AXIS2_PLACEMENT_3D ( 'NONE', #45928, #114018, #76015 ) ;
#63973=DIRECTION ( 'NONE',  ( 0.000000000000000000, 1.000000000000000000, 0.000000000000000000 ) ) ;
#63974=CARTESIAN_POINT ( 'NONE',  ( 9.999999999999948486, 2.500000000000000000, -4.230127018922201998 ) ) ;
#63975=VERTEX_POINT ( 'NONE', #124528 ) ;
#63976=ORIENTED_EDGE ( 'NONE', *, *, #111922, .T. ) ;
#63977=CARTESIAN_POINT ( 'NONE',  ( 7.049999999999930544, 2.500000000000000000, -6.495190528383302464 ) ) ;
#63978=VERTEX_POINT ( 'NONE', #122589 ) ;
#63979=CARTESIAN_POINT ( 'NONE',  ( 7.499999999999927169, 2.500000000000000000, -5.022947341949754119 ) ) ;
#63981=VERTEX_POINT ( 'NONE', #14543 ) ;
#63982=DIRECTION ( 'NONE',  ( 0.000000000000000000, 1.000000000000000000, 0.000000000000000000 ) ) ;
#63983=DIRECTION ( 'NONE',  ( -0.000000000000000000, 1.000000000000000000, -0.000000000000000000 ) ) ;
#63984=DIRECTION ( 'NONE',  ( 0.000000000000000000, 0.000000000000000000, -1.000000000000000000 ) ) ;
#63985=CARTESIAN_POINT ( 'NONE',  ( -11.89999999999999680, 12.50000000000000000, -4.676537180435976104 ) ) ;
#63986=VERTEX_POINT ( 'NONE', #84594 ) ;
#63987=CARTESIAN_POINT ( 'NONE',  ( -3.350000000000031619, 12.50000000000000000, -5.802370205355749988 ) ) ;
#63988=CIRCLE ( 'NONE', #34760, 0.06509327318403743123 ) ;
#63989=CIRCLE ( 'NONE', #59825, 0.06509327318403741736 ) ;
#63990=CARTESIAN_POINT ( 'NONE',  ( 43.31214921609998925, -3.511364963944068940, 3.941696051831963032 ) ) ;
#63991=ORIENTED_EDGE ( 'NONE', *, *, #87974, .F. ) ;
#63992=EDGE_LOOP ( 'NONE', ( #53715, #51960 ) ) ;
#63995=DIRECTION ( 'NONE',  ( 0.000000000000000000, 1.000000000000000000, 0.000000000000000000 ) ) ;
#63996=DIRECTION ( 'NONE',  ( 0.000000000000000000, 0.000000000000000000, -1.000000000000000000 ) ) ;
#63997=DIRECTION ( 'NONE',  ( 0.000000000000000000, 1.000000000000000000, 0.000000000000000000 ) ) ;
#63998=AXIS2_PLACEMENT_3D ( 'NONE', #118105, #49394, #97184 ) ;
#63999=DIRECTION ( 'NONE',  ( -0.000000000000000000, -1.000000000000000000, -0.000000000000000000 ) ) ;
#64000=CIRCLE ( 'NONE', #28499, 0.1000000000000000472 ) ;
#64001=EDGE_CURVE ( 'NONE', #82140, #122182, #34221, .T. ) ;
#64002=DIRECTION ( 'NONE',  ( 0.000000000000000000, 1.000000000000000000, 0.000000000000000000 ) ) ;
#64003=CARTESIAN_POINT ( 'NONE',  ( -7.500000000000001776, 2.500000000000000000, 1.734723475976807094E-15 ) ) ;
#64004=FACE_OUTER_BOUND ( 'NONE', #96829, .T. ) ;
#64005=DIRECTION ( 'NONE',  ( 0.000000000000000000, 0.000000000000000000, 1.000000000000000000 ) ) ;
#64007=DIRECTION ( 'NONE',  ( 0.000000000000000000, 0.000000000000000000, 1.000000000000000000 ) ) ;
#64008=EDGE_CURVE ( 'NONE', #7770, #93441, #10295, .T. ) ;
#64009=ORIENTED_EDGE ( 'NONE', *, *, #107595, .T. ) ;
#64011=AXIS2_PLACEMENT_3D ( 'NONE', #1337, #9239, #693 ) ;
#64012=ORIENTED_EDGE ( 'NONE', *, *, #94508, .T. ) ;
#64013=EDGE_CURVE ( 'NONE', #32792, #123530, #98112, .T. ) ;
#64014=ORIENTED_EDGE ( 'NONE', *, *, #88398, .F. ) ;
#64015=EDGE_CURVE ( 'NONE', #20221, #50581, #68862, .T. ) ;
#64016=CARTESIAN_POINT ( 'NONE',  ( 11.24999999999990941, 2.500000000000000000, -1.472243186433550122 ) ) ;
#64017=DIRECTION ( 'NONE',  ( -0.000000000000000000, -1.000000000000000000, -0.000000000000000000 ) ) ;
#64018=EDGE_LOOP ( 'NONE', ( #17759, #14801 ) ) ;
#64019=CARTESIAN_POINT ( 'NONE',  ( -12.89999999999999147, 12.50000000000000000, 3.702399969078682407 ) ) ;
#64020=ADVANCED_FACE ( 'NONE', ( #34872 ), #123237, .T. ) ;
#64021=PLANE ( 'NONE',  #15681 ) ;
#64022=DIRECTION ( 'NONE',  ( -0.000000000000000000, 1.000000000000000000, -0.000000000000000000 ) ) ;
#64023=VERTEX_POINT ( 'NONE', #94398 ) ;
#64024=EDGE_CURVE ( 'NONE', #23353, #115231, #21821, .T. ) ;
#64025=DIRECTION ( 'NONE',  ( -0.000000000000000000, -1.000000000000000000, -0.000000000000000000 ) ) ;
#64026=CONICAL_SURFACE ( 'NONE', #126723, 0.1000000000000002554, 0.003490658503988666988 ) ;
#64027=DIRECTION ( 'NONE',  ( 0.000000000000000000, 0.000000000000000000, 1.000000000000000000 ) ) ;
#64028=ORIENTED_EDGE ( 'NONE', *, *, #34481, .T. ) ;
#64029=AXIS2_PLACEMENT_3D ( 'NONE', #118075, #66397, #106330 ) ;
#64030=ORIENTED_EDGE ( 'NONE', *, *, #28612, .F. ) ;
#64031=VERTEX_POINT ( 'NONE', #52552 ) ;
#64032=ORIENTED_EDGE ( 'NONE', *, *, #109572, .F. ) ;
#64033=CARTESIAN_POINT ( 'NONE',  ( 5.399999999999935518, 12.50000000000000000, -4.330127018922201643 ) ) ;
#64034=AXIS2_PLACEMENT_3D ( 'NONE', #51549, #110444, #41094 ) ;
#64035=CARTESIAN_POINT ( 'NONE',  ( 4.349999999999939249, 12.50000000000000000, 2.446380397790835826 ) ) ;
#64036=DIRECTION ( 'NONE',  ( 0.000000000000000000, 0.000000000000000000, 1.000000000000000000 ) ) ;
#64037=VECTOR ( 'NONE', #51858, 1000.000000000000000 ) ;
#64038=DIRECTION ( 'NONE',  ( 0.000000000000000000, 0.000000000000000000, 1.000000000000000000 ) ) ;
#64039=VERTEX_POINT ( 'NONE', #61751 ) ;
#64040=CIRCLE ( 'NONE', #9754, 0.06509327318403745899 ) ;
#64041=DIRECTION ( 'NONE',  ( -0.000000000000000000, -1.000000000000000000, -0.000000000000000000 ) ) ;
#64042=VERTEX_POINT ( 'NONE', #121942 ) ;
#64043=CARTESIAN_POINT ( 'NONE',  ( -6.250000000000019540, 2.500000000000000000, -2.857883832488653741 ) ) ;
#64044=CARTESIAN_POINT ( 'NONE',  ( 12.06068301339626281, -1.499999999999807931, -8.632777000277656043 ) ) ;
#64045=CARTESIAN_POINT ( 'NONE',  ( -3.750000000000026201, 2.500000000000000000, 5.702370205355745014 ) ) ;
#64046=CARTESIAN_POINT ( 'NONE',  ( 17.17161331427274007, -0.4678040054248471802, 5.513957101008608142 ) ) ;
#64047=CIRCLE ( 'NONE', #7602, 0.06509327318403745899 ) ;
#64048=ORIENTED_EDGE ( 'NONE', *, *, #42693, .T. ) ;
#64049=ADVANCED_FACE ( 'NONE', ( #4713 ), #111464, .T. ) ;
#64050=CIRCLE ( 'NONE', #62006, 0.06509327318403745899 ) ;
#64051=ORIENTED_EDGE ( 'NONE', *, *, #3600, .F. ) ;
#64052=ORIENTED_EDGE ( 'NONE', *, *, #51221, .T. ) ;
#64053=CARTESIAN_POINT ( 'NONE',  ( 9.549999999999918998, 2.500000000000000000, 2.065063509461097624 ) ) ;
#64054=CARTESIAN_POINT ( 'NONE',  ( 7.699999999999925571, 2.500000000000000000, 4.083716857408420609 ) ) ;
#64055=FACE_OUTER_BOUND ( 'NONE', #120618, .T. ) ;
#64056=FACE_BOUND ( 'NONE', #23847, .T. ) ;
#64057=CARTESIAN_POINT ( 'NONE',  ( -6.050000000000017586, 12.50000000000000000, 6.083687093685482772 ) ) ;
#64058=CARTESIAN_POINT ( 'NONE',  ( 6.449999999999930012, 12.50000000000000000, 6.776507416713035248 ) ) ;
#64059=EDGE_CURVE ( 'NONE', #9579, #118717, #52153, .T. ) ;
#64060=DIRECTION ( 'NONE',  ( 0.000000000000000000, 0.000000000000000000, 1.000000000000000000 ) ) ;
#64061=EDGE_CURVE ( 'NONE', #55669, #15992, #100180, .T. ) ;
#64063=CARTESIAN_POINT ( 'NONE',  ( -6.650000000000018119, 2.500000000000000000, -7.088010851410853519 ) ) ;
#64064=EDGE_CURVE ( 'NONE', #18602, #112155, #106431, .T. ) ;
#64065=DIRECTION ( 'NONE',  ( 0.000000000000000000, 0.000000000000000000, 1.000000000000000000 ) ) ;
#64066=VERTEX_POINT ( 'NONE', #32304 ) ;
#64067=EDGE_CURVE ( 'NONE', #181, #31627, #60492, .T. ) ;
#64068=DIRECTION ( 'NONE',  ( 0.000000000000000000, 0.000000000000000000, 1.000000000000000000 ) ) ;
#64069=EDGE_CURVE ( 'NONE', #125139, #56994, #6161, .T. ) ;
#64070=EDGE_LOOP ( 'NONE', ( #108612, #115383 ) ) ;
#64071=ORIENTED_EDGE ( 'NONE', *, *, #39833, .F. ) ;
#64072=ORIENTED_EDGE ( 'NONE', *, *, #40565, .T. ) ;
#64074=CARTESIAN_POINT ( 'NONE',  ( -3.950000000000028155, 2.500000000000000000, -6.841600689897077814 ) ) ;
#64075=FACE_BOUND ( 'NONE', #50165, .T. ) ;
#64076=DIRECTION ( 'NONE',  ( 0.000000000000000000, 0.000000000000000000, -1.000000000000000000 ) ) ;
#64077=EDGE_CURVE ( 'NONE', #113211, #64031, #57047, .T. ) ;
#64078=ADVANCED_FACE ( 'NONE', ( #16472 ), #55772, .T. ) ;
#64079=CIRCLE ( 'NONE', #16031, 0.06509327318403745899 ) ;
#64080=CIRCLE ( 'NONE', #43173, 0.06509327318403745899 ) ;
#64081=ORIENTED_EDGE ( 'NONE', *, *, #126674, .F. ) ;
#64082=LINE ( 'NONE', #104010, #17458 ) ;
#64083=CARTESIAN_POINT ( 'NONE',  ( -10.60000000000000320, 2.500000000000000000, -4.776537180435973085 ) ) ;
#64084=ORIENTED_EDGE ( 'NONE', *, *, #110301, .T. ) ;
#64085=CARTESIAN_POINT ( 'NONE',  ( 7.899999999999923084, 2.500000000000000000, 0.6928203230275494784 ) ) ;
#64086=DIRECTION ( 'NONE',  ( -0.000000000000000000, -1.000000000000000000, -0.000000000000000000 ) ) ;
#64087=AXIS2_PLACEMENT_3D ( 'NONE', #72254, #914, #80125 ) ;
#64088=ORIENTED_EDGE ( 'NONE', *, *, #16186, .F. ) ;
#64089=DIRECTION ( 'NONE',  ( 0.000000000000000000, 0.000000000000000000, 1.000000000000000000 ) ) ;
#64090=DIRECTION ( 'NONE',  ( 0.000000000000000000, 1.000000000000000000, 0.000000000000000000 ) ) ;
#64091=CONICAL_SURFACE ( 'NONE', #43186, 0.1000000000000000472, 0.003490658503988666988 ) ;
#64092=CIRCLE ( 'NONE', #18022, 0.1000000000000002554 ) ;
#64093=ORIENTED_EDGE ( 'NONE', *, *, #45305, .T. ) ;
#64094=AXIS2_PLACEMENT_3D ( 'NONE', #27410, #107276, #96800 ) ;
#64095=LINE ( 'NONE', #85017, #57273 ) ;
#64096=CARTESIAN_POINT ( 'NONE',  ( 13.14999999999989733, 2.500000000000000000, -1.818653347947325916 ) ) ;
#64097=CARTESIAN_POINT ( 'NONE',  ( -1.250000000000001110, 2.500000000000000000, -6.495190528383302464 ) ) ;
#64098=ORIENTED_EDGE ( 'NONE', *, *, #125202, .T. ) ;
#64099=ORIENTED_EDGE ( 'NONE', *, *, #88293, .T. ) ;
#64100=CARTESIAN_POINT ( 'NONE',  ( 11.24999999999994316, 12.50000000000000000, -6.495190528383302464 ) ) ;
#64101=EDGE_LOOP ( 'NONE', ( #97086, #65857, #33515, #86206 ) ) ;
#64102=CARTESIAN_POINT ( 'NONE',  ( -2.500000000000030642, 2.500000000000000000, -4.922947341949753586 ) ) ;
#64103=CARTESIAN_POINT ( 'NONE',  ( -3.950000000000026379, 12.50000000000000000, 6.841600689897072485 ) ) ;
#64104=ORIENTED_EDGE ( 'NONE', *, *, #96284, .T. ) ;
#64105=CARTESIAN_POINT ( 'NONE',  ( 14.59999999999989484, 12.50000000000000000, 0.06509327318403515528 ) ) ;
#64106=CARTESIAN_POINT ( 'NONE',  ( -9.150000000000005684, 2.500000000000000000, 5.902370205355745192 ) ) ;
#64107=DIRECTION ( 'NONE',  ( -0.000000000000000000, -1.000000000000000000, -0.000000000000000000 ) ) ;
#64108=LINE ( 'NONE', #26769, #86288 ) ;
#64109=CIRCLE ( 'NONE', #70379, 0.06509327318403745899 ) ;
#64111=VECTOR ( 'NONE', #46080, 1000.000000000000000 ) ;
#64112=EDGE_LOOP ( 'NONE', ( #55745, #35850 ) ) ;
#64113=EDGE_CURVE ( 'NONE', #104184, #98077, #58424, .T. ) ;
#64114=ORIENTED_EDGE ( 'NONE', *, *, #47799, .T. ) ;
#64115=DIRECTION ( 'NONE',  ( 0.000000000000000000, 1.000000000000000000, 0.000000000000000000 ) ) ;
#64116=CIRCLE ( 'NONE', #103836, 0.1000000000000002554 ) ;
#64117=CARTESIAN_POINT ( 'NONE',  ( -6.850000000000017408, 12.50000000000000000, -6.213873640053564351 ) ) ;
#64118=CARTESIAN_POINT ( 'NONE',  ( 5.649999999999934630, 2.500000000000000000, -2.611473670974877592 ) ) ;
#64119=ORIENTED_EDGE ( 'NONE', *, *, #13359, .F. ) ;
#64120=ORIENTED_EDGE ( 'NONE', *, *, #84372, .F. ) ;
#64122=FACE_OUTER_BOUND ( 'NONE', #119932, .T. ) ;
#64123=AXIS2_PLACEMENT_3D ( 'NONE', #36420, #107058, #8220 ) ;
#64124=AXIS2_PLACEMENT_3D ( 'NONE', #44606, #83253, #67941 ) ;
#64125=CARTESIAN_POINT ( 'NONE',  ( -2.050000000000033129, 12.50000000000000000, 2.099970236277060032 ) ) ;
#64126=DIRECTION ( 'NONE',  ( 0.000000000000000000, 0.000000000000000000, 1.000000000000000000 ) ) ;
#64128=CARTESIAN_POINT ( 'NONE',  ( 10.39999999999990976, 12.50000000000000000, -4.330127018922201643 ) ) ;
#64129=DIRECTION ( 'NONE',  ( 0.000000000000000000, 0.000000000000000000, 1.000000000000000000 ) ) ;
#64130=CARTESIAN_POINT ( 'NONE',  ( -6.900000000000019007, 12.50000000000000000, -4.676537180435978769 ) ) ;
#64131=PLANE ( 'NONE',  #13144 ) ;
#64132=VECTOR ( 'NONE', #100802, 1000.000000000000000 ) ;
#64133=PLANE ( 'NONE',  #74916 ) ;
#64134=CIRCLE ( 'NONE', #5544, 0.06509327318403745899 ) ;
#64135=ORIENTED_EDGE ( 'NONE', *, *, #6673, .F. ) ;
#64136=VECTOR ( 'NONE', #115629, 1000.000000000000000 ) ;
#64137=AXIS2_PLACEMENT_3D ( 'NONE', #74721, #117844, #127053 ) ;
#64138=DIRECTION ( 'NONE',  ( 0.000000000000000000, 0.000000000000000000, 1.000000000000000000 ) ) ;
#64139=VERTEX_POINT ( 'NONE', #6630 ) ;
#64140=ORIENTED_EDGE ( 'NONE', *, *, #93356, .T. ) ;
#64141=DIRECTION ( 'NONE',  ( -0.000000000000000000, -1.000000000000000000, -0.000000000000000000 ) ) ;
#64142=DIRECTION ( 'NONE',  ( 0.000000000000000000, 1.000000000000000000, 0.000000000000000000 ) ) ;
#64143=FACE_OUTER_BOUND ( 'NONE', #51369, .T. ) ;
#64144=DIRECTION ( 'NONE',  ( -0.000000000000000000, 1.000000000000000000, -0.000000000000000000 ) ) ;
#64145=CARTESIAN_POINT ( 'NONE',  ( 9.349999999999919709, 2.500000000000000000, -6.148780366869526226 ) ) ;
#64146=PLANE ( 'NONE',  #51117 ) ;
#64147=CARTESIAN_POINT ( 'NONE',  ( 11.64999999999990798, 2.500000000000000000, -2.857883832488653741 ) ) ;
#64148=EDGE_LOOP ( 'NONE', ( #7535, #84839 ) ) ;
#64149=CARTESIAN_POINT ( 'NONE',  ( 5.849999999999933920, 2.500000000000000000, -2.857883832488653741 ) ) ;
#64150=AXIS2_PLACEMENT_3D ( 'NONE', #84875, #93413, #124811 ) ;
#64151=DIRECTION ( 'NONE',  ( -4.274815082592931898E-19, -0.9999939076577903929, -0.003490651415223739937 ) ) ;
#64153=EDGE_CURVE ( 'NONE', #66867, #49607, #50032, .T. ) ;
#64154=ORIENTED_EDGE ( 'NONE', *, *, #117203, .F. ) ;
#64155=ORIENTED_EDGE ( 'NONE', *, *, #113078, .F. ) ;
#64156=EDGE_CURVE ( 'NONE', #3522, #98275, #87156, .T. ) ;
#64157=VERTEX_POINT ( 'NONE', #15179 ) ;
#64158=EDGE_CURVE ( 'NONE', #35476, #56841, #112800, .T. ) ;
#64159=LINE ( 'NONE', #94264, #71320 ) ;
#64160=DIRECTION ( 'NONE',  ( 0.000000000000000000, 0.000000000000000000, -1.000000000000000000 ) ) ;
#64161=CONICAL_SURFACE ( 'NONE', #60078, 0.1000000000000002554, 0.003490658503988666988 ) ;
#64163=CIRCLE ( 'NONE', #22432, 0.1000000000000002554 ) ;
#64164=DIRECTION ( 'NONE',  ( -4.274815082592931898E-19, -0.9999939076577903929, -0.003490651415223739937 ) ) ;
#64165=ADVANCED_FACE ( 'NONE', ( #65590 ), #1961, .T. ) ;
#64166=DIRECTION ( 'NONE',  ( 0.000000000000000000, -0.000000000000000000, 1.000000000000000000 ) ) ;
#64167=EDGE_CURVE ( 'NONE', #87148, #77466, #47952, .T. ) ;
#64168=ORIENTED_EDGE ( 'NONE', *, *, #48710, .F. ) ;
#64169=DIRECTION ( 'NONE',  ( 0.000000000000000000, 1.000000000000000000, 0.000000000000000000 ) ) ;
#64170=EDGE_CURVE ( 'NONE', #5316, #61065, #27021, .T. ) ;
#64171=EDGE_CURVE ( 'NONE', #111830, #21908, #43762, .T. ) ;
#64172=DIRECTION ( 'NONE',  ( 0.000000000000000000, 0.000000000000000000, 1.000000000000000000 ) ) ;
#64173=AXIS2_PLACEMENT_3D ( 'NONE', #87688, #16350, #17660 ) ;
#64174=VECTOR ( 'NONE', #32660, 1000.000000000000000 ) ;
#64175=FACE_OUTER_BOUND ( 'NONE', #18632, .T. ) ;
#64177=EDGE_LOOP ( 'NONE', ( #2747, #126235 ) ) ;
#64178=EDGE_LOOP ( 'NONE', ( #545, #85303 ) ) ;
#64179=DIRECTION ( 'NONE',  ( 0.000000000000000000, 0.000000000000000000, 1.000000000000000000 ) ) ;
#64180=CIRCLE ( 'NONE', #24479, 0.06509327318403745899 ) ;
#64181=VECTOR ( 'NONE', #81763, 1000.000000000000000 ) ;
#64182=CARTESIAN_POINT ( 'NONE',  ( -8.350000000000013856, 12.50000000000000000, -2.165063509461101710 ) ) ;
#64183=DIRECTION ( 'NONE',  ( -4.274815082592931898E-19, -0.9999939076577903929, -0.003490651415223739937 ) ) ;
#64184=CIRCLE ( 'NONE', #51685, 0.06509327318403745899 ) ;
#64185=ORIENTED_EDGE ( 'NONE', *, *, #86303, .F. ) ;
#64186=CARTESIAN_POINT ( 'NONE',  ( -6.249999999999981348, 2.500000000000000000, 2.165063509461097713 ) ) ;
#64187=CARTESIAN_POINT ( 'NONE',  ( 0.8499999999999553468, 2.500000000000000000, -2.165063509461101710 ) ) ;
#64188=CARTESIAN_POINT ( 'NONE',  ( 0.3999999999999568345, 2.500000000000000000, -4.922947341949753586 ) ) ;
#64189=DIRECTION ( 'NONE',  ( 0.000000000000000000, -0.9999939076577903929, 0.003490651415223739937 ) ) ;
#64190=DIRECTION ( 'NONE',  ( -0.000000000000000000, 1.000000000000000000, -0.000000000000000000 ) ) ;
#64191=EDGE_LOOP ( 'NONE', ( #83324, #49581, #119621, #34348 ) ) ;
#64192=ORIENTED_EDGE ( 'NONE', *, *, #12849, .F. ) ;
#64193=EDGE_CURVE ( 'NONE', #47717, #56128, #104381, .T. ) ;
#64195=DIRECTION ( 'NONE',  ( 0.000000000000000000, -0.9999939076577903929, 0.003490651415223739937 ) ) ;
#64196=CONICAL_SURFACE ( 'NONE', #32831, 0.09999999999999982514, 0.003490658503988666988 ) ;
#64197=DIRECTION ( 'NONE',  ( 0.000000000000000000, 0.000000000000000000, -1.000000000000000000 ) ) ;
#64198=DIRECTION ( 'NONE',  ( 0.000000000000000000, 0.000000000000000000, 1.000000000000000000 ) ) ;
#64199=AXIS2_PLACEMENT_3D ( 'NONE', #52509, #20489, #31594 ) ;
#64200=CARTESIAN_POINT ( 'NONE',  ( -9.999999999999969802, 2.500000000000000000, 4.330127018922196314 ) ) ;
#64201=EDGE_LOOP ( 'NONE', ( #95366, #120006 ) ) ;
#64202=CONICAL_SURFACE ( 'NONE', #43301, 0.09999999999999982514, 0.003490658503988666988 ) ;
#64203=ADVANCED_FACE ( 'NONE', ( #57719 ), #24955, .T. ) ;
#64204=EDGE_LOOP ( 'NONE', ( #42901, #87381, #78099, #115431 ) ) ;
#64205=EDGE_CURVE ( 'NONE', #104031, #2125, #81413, .T. ) ;
#64206=DIRECTION ( 'NONE',  ( 0.000000000000000000, -0.000000000000000000, 1.000000000000000000 ) ) ;
#64207=CARTESIAN_POINT ( 'NONE',  ( 11.24999999999994493, 12.50000000000000000, 6.495190528383297135 ) ) ;
#64208=CONICAL_SURFACE ( 'NONE', #7774, 0.09999999999999982514, 0.003490658503988666988 ) ;
#64209=CARTESIAN_POINT ( 'NONE',  ( 18.00406199218826231, -1.510509990051560170, -4.944015969580405567 ) ) ;
#64210=EDGE_CURVE ( 'NONE', #78150, #33245, #113110, .T. ) ;
#64211=CIRCLE ( 'NONE', #11984, 0.1000000000000002554 ) ;
#64212=FACE_OUTER_BOUND ( 'NONE', #69718, .T. ) ;
#64213=VERTEX_POINT ( 'NONE', #7953 ) ;
#64214=DIRECTION ( 'NONE',  ( 0.000000000000000000, 0.000000000000000000, -1.000000000000000000 ) ) ;
#64215=AXIS2_PLACEMENT_3D ( 'NONE', #74653, #93658, #24915 ) ;
#64216=CARTESIAN_POINT ( 'NONE',  ( 8.349999999999923261, 12.50000000000000000, -7.188010851410854052 ) ) ;
#64217=EDGE_CURVE ( 'NONE', #99657, #53810, #92177, .T. ) ;
#64218=ORIENTED_EDGE ( 'NONE', *, *, #109906, .T. ) ;
#64219=DIRECTION ( 'NONE',  ( -0.000000000000000000, 1.000000000000000000, -0.000000000000000000 ) ) ;
#64220=AXIS2_PLACEMENT_3D ( 'NONE', #52861, #80398, #22134 ) ;
#64221=EDGE_CURVE ( 'NONE', #2505, #87803, #73393, .T. ) ;
#64222=ORIENTED_EDGE ( 'NONE', *, *, #52692, .F. ) ;
#64223=DIRECTION ( 'NONE',  ( 0.000000000000000000, 1.000000000000000000, 0.000000000000000000 ) ) ;
#64224=EDGE_CURVE ( 'NONE', #15992, #55669, #46213, .T. ) ;
#64225=EDGE_CURVE ( 'NONE', #54758, #20844, #86512, .T. ) ;
#64226=CIRCLE ( 'NONE', #101888, 0.1000000000000002554 ) ;
#64228=EDGE_LOOP ( 'NONE', ( #99371, #13278, #22643, #47350 ) ) ;
#64229=CARTESIAN_POINT ( 'NONE',  ( -5.400000000000024336, 12.50000000000000000, -3.572213422710612374 ) ) ;
#64230=DIRECTION ( 'NONE',  ( 0.000000000000000000, 0.000000000000000000, -1.000000000000000000 ) ) ;
#64231=ORIENTED_EDGE ( 'NONE', *, *, #66093, .T. ) ;
#64232=ORIENTED_EDGE ( 'NONE', *, *, #38028, .F. ) ;
#64234=DIRECTION ( 'NONE',  ( 0.000000000000000000, 1.000000000000000000, 0.000000000000000000 ) ) ;
#64235=EDGE_CURVE ( 'NONE', #49584, #81973, #25266, .T. ) ;
#64236=CARTESIAN_POINT ( 'NONE',  ( 2.899999999999946620, 12.50000000000000000, -3.637306695894650055 ) ) ;
#64237=DIRECTION ( 'NONE',  ( 0.000000000000000000, 0.000000000000000000, 1.000000000000000000 ) ) ;
#64238=DIRECTION ( 'NONE',  ( -0.000000000000000000, 1.000000000000000000, -0.000000000000000000 ) ) ;
#64239=LINE ( 'NONE', #74063, #128346 ) ;
#64240=DIRECTION ( 'NONE',  ( 0.000000000000000000, 0.000000000000000000, 1.000000000000000000 ) ) ;
#64241=CARTESIAN_POINT ( 'NONE',  ( -11.24999999999999822, 12.50000000000000000, 1.407149913249508000 ) ) ;
#64242=VERTEX_POINT ( 'NONE', #59672 ) ;
#64243=ORIENTED_EDGE ( 'NONE', *, *, #55463, .F. ) ;
#64244=CARTESIAN_POINT ( 'NONE',  ( -0.6500000000000403233, 2.500000000000000000, 1.818653347947321475 ) ) ;
#64245=DIRECTION ( 'NONE',  ( 0.000000000000000000, 0.000000000000000000, -1.000000000000000000 ) ) ;
#64246=CARTESIAN_POINT ( 'NONE',  ( -5.200000000000024158, 2.500000000000000000, -4.576537180435977348 ) ) ;
#64247=ORIENTED_EDGE ( 'NONE', *, *, #22845, .T. ) ;
#64248=EDGE_LOOP ( 'NONE', ( #115993, #38735, #31891, #6675 ) ) ;
#64249=CARTESIAN_POINT ( 'NONE',  ( -1.900000000000034550, 12.50000000000000000, 4.741630453620009789 ) ) ;
#64250=EDGE_LOOP ( 'NONE', ( #43392, #113822 ) ) ;
#64251=CARTESIAN_POINT ( 'NONE',  ( -11.25000000000000000, 12.50000000000000000, 7.188010851410848723 ) ) ;
#64252=CARTESIAN_POINT ( 'NONE',  ( 17.50000000000000000, -2.500000000000000000, 2.922290670089274567 ) ) ;
#64253=ORIENTED_EDGE ( 'NONE', *, *, #114875, .F. ) ;
#64254=DIRECTION ( 'NONE',  ( -4.274815082592931898E-19, -0.9999939076577903929, -0.003490651415223739937 ) ) ;
#64255=CARTESIAN_POINT ( 'NONE',  ( -8.100000000000013856, 12.50000000000000000, -4.048810130592463530 ) ) ;
#64256=AXIS2_PLACEMENT_3D ( 'NONE', #97774, #118051, #118698 ) ;
#64257=DIRECTION ( 'NONE',  ( -0.000000000000000000, -1.000000000000000000, -0.000000000000000000 ) ) ;
#64258=CIRCLE ( 'NONE', #1560, 0.1000000000000002554 ) ;
#64259=PLANE ( 'NONE',  #61266 ) ;
#64260=DIRECTION ( 'NONE',  ( -0.000000000000000000, 1.000000000000000000, -0.000000000000000000 ) ) ;
#64261=CARTESIAN_POINT ( 'NONE',  ( -11.25000000000000000, 2.500000000000000000, 2.957883832488649389 ) ) ;
#64263=PLANE ( 'NONE',  #59035 ) ;
#64264=CARTESIAN_POINT ( 'NONE',  ( -4.999999999999986677, 2.500000000000000000, -2.276824562219559311E-15 ) ) ;
#64265=VECTOR ( 'NONE', #14282, 1000.000000000000000 ) ;
#64266=CIRCLE ( 'NONE', #112865, 0.06509327318403745899 ) ;
#64268=ORIENTED_EDGE ( 'NONE', *, *, #46810, .T. ) ;
#64270=EDGE_CURVE ( 'NONE', #8618, #3902, #91035, .T. ) ;
#64271=ORIENTED_EDGE ( 'NONE', *, *, #29648, .T. ) ;
#64272=CARTESIAN_POINT ( 'NONE',  ( 10.84999999999991260, 12.50000000000000000, 7.253104124594885960 ) ) ;
#64273=ORIENTED_EDGE ( 'NONE', *, *, #91656, .T. ) ;
#64274=VERTEX_POINT ( 'NONE', #108086 ) ;
#64275=ORIENTED_EDGE ( 'NONE', *, *, #24080, .T. ) ;
#64276=ORIENTED_EDGE ( 'NONE', *, *, #80337, .T. ) ;
#64277=DIRECTION ( 'NONE',  ( 0.000000000000000000, -0.000000000000000000, 1.000000000000000000 ) ) ;
#64278=CIRCLE ( 'NONE', #101662, 0.1000000000000002554 ) ;
#64279=VECTOR ( 'NONE', #30767, 1000.000000000000000 ) ;
#64280=CONICAL_SURFACE ( 'NONE', #89327, 0.09999999999999982514, 0.003490658503988666988 ) ;
#64281=PLANE ( 'NONE',  #44682 ) ;
#64282=CARTESIAN_POINT ( 'NONE',  ( -0.6500000000000389910, 2.500000000000000000, -1.718653347947326049 ) ) ;
#64283=DIRECTION ( 'NONE',  ( 0.000000000000000000, 0.000000000000000000, -1.000000000000000000 ) ) ;
#64284=DIRECTION ( 'NONE',  ( 0.000000000000000000, -0.9999939076577903929, 0.003490651415223739937 ) ) ;
#64285=EDGE_CURVE ( 'NONE', #127796, #113021, #87959, .T. ) ;
#64286=VERTEX_POINT ( 'NONE', #77990 ) ;
#64287=DIRECTION ( 'NONE',  ( -0.000000000000000000, 1.000000000000000000, -0.000000000000000000 ) ) ;
#64288=EDGE_LOOP ( 'NONE', ( #46448, #58999 ) ) ;
#64289=AXIS2_PLACEMENT_3D ( 'NONE', #34340, #74245, #91099 ) ;
#64290=ORIENTED_EDGE ( 'NONE', *, *, #42449, .F. ) ;
#64291=ORIENTED_EDGE ( 'NONE', *, *, #37490, .T. ) ;
#64292=AXIS2_PLACEMENT_3D ( 'NONE', #17241, #24519, #106925 ) ;
#64293=DIRECTION ( 'NONE',  ( -0.000000000000000000, 1.000000000000000000, -0.000000000000000000 ) ) ;
#64294=EDGE_LOOP ( 'NONE', ( #81982, #60462, #27925, #42223 ) ) ;
#64295=ORIENTED_EDGE ( 'NONE', *, *, #3194, .F. ) ;
#64296=ORIENTED_EDGE ( 'NONE', *, *, #89048, .T. ) ;
#64297=AXIS2_PLACEMENT_3D ( 'NONE', #104994, #80387, #15322 ) ;
#64298=CONICAL_SURFACE ( 'NONE', #85230, 0.09999999999999982514, 0.003490658503988666988 ) ;
#64300=DIRECTION ( 'NONE',  ( 0.000000000000000000, 0.000000000000000000, 1.000000000000000000 ) ) ;
#64301=DIRECTION ( 'NONE',  ( 0.000000000000000000, 1.000000000000000000, 0.000000000000000000 ) ) ;
#64302=AXIS2_PLACEMENT_3D ( 'NONE', #44886, #44213, #104433 ) ;
#64303=DIRECTION ( 'NONE',  ( -0.000000000000000000, 1.000000000000000000, -0.000000000000000000 ) ) ;
#64304=DIRECTION ( 'NONE',  ( -0.000000000000000000, -1.000000000000000000, -0.000000000000000000 ) ) ;
#64305=DIRECTION ( 'NONE',  ( -0.000000000000000000, 1.000000000000000000, -0.000000000000000000 ) ) ;
#64306=CIRCLE ( 'NONE', #110369, 0.09999999999999999167 ) ;
#64307=DIRECTION ( 'NONE',  ( -0.000000000000000000, -1.000000000000000000, -0.000000000000000000 ) ) ;
#64308=CIRCLE ( 'NONE', #5796, 0.06509327318403745899 ) ;
#64309=VERTEX_POINT ( 'NONE', #89104 ) ;
#64310=AXIS2_PLACEMENT_3D ( 'NONE', #27317, #16835, #105252 ) ;
#64311=CARTESIAN_POINT ( 'NONE',  ( 8.949999999999915801, 2.500000000000000000, -1.818653347947326138 ) ) ;
#64312=EDGE_CURVE ( 'NONE', #43648, #96511, #49838, .T. ) ;
#64313=VERTEX_POINT ( 'NONE', #80580 ) ;
#64314=CARTESIAN_POINT ( 'NONE',  ( 2.499999999999983569, 12.50000000000000000, -2.276824562219559311E-15 ) ) ;
#64315=VERTEX_POINT ( 'NONE', #40012 ) ;
#64316=AXIS2_PLACEMENT_3D ( 'NONE', #114350, #14832, #94707 ) ;
#64317=ORIENTED_EDGE ( 'NONE', *, *, #66857, .F. ) ;
#64319=CARTESIAN_POINT ( 'NONE',  ( 7.499999999999923617, 2.500000000000000000, 0.7928203230275495672 ) ) ;
#64320=DIRECTION ( 'NONE',  ( 0.000000000000000000, 0.000000000000000000, -1.000000000000000000 ) ) ;
#64322=AXIS2_PLACEMENT_3D ( 'NONE', #37075, #37710, #19337 ) ;
#64323=CARTESIAN_POINT ( 'NONE',  ( -9.600000000000006750, 2.500000000000000000, 3.637306695894644726 ) ) ;
#64324=ORIENTED_EDGE ( 'NONE', *, *, #49751, .F. ) ;
#64325=EDGE_CURVE ( 'NONE', #38043, #96705, #6467, .T. ) ;
#64326=LINE ( 'NONE', #55159, #15689 ) ;
#64327=EDGE_CURVE ( 'NONE', #118169, #18418, #79662, .T. ) ;
#64328=ORIENTED_EDGE ( 'NONE', *, *, #36335, .F. ) ;
#64330=CARTESIAN_POINT ( 'NONE',  ( -0.8000000000000381251, 2.500000000000000000, 4.230127018922196669 ) ) ;
#64331=FACE_OUTER_BOUND ( 'NONE', #72729, .T. ) ;
#64332=EDGE_CURVE ( 'NONE', #103079, #100426, #75453, .T. ) ;
#64333=FACE_OUTER_BOUND ( 'NONE', #42830, .T. ) ;
#64334=EDGE_CURVE ( 'NONE', #35473, #92869, #60924, .T. ) ;
#64335=ADVANCED_FACE ( 'NONE', ( #100835 ), #104693, .T. ) ;
#64336=DIRECTION ( 'NONE',  ( 0.000000000000000000, 0.000000000000000000, 1.000000000000000000 ) ) ;
#64337=DIRECTION ( 'NONE',  ( 0.000000000000000000, -0.9999939076577903929, 0.003490651415223739937 ) ) ;
#64338=EDGE_LOOP ( 'NONE', ( #2209, #126666 ) ) ;
#64339=EDGE_CURVE ( 'NONE', #41615, #42781, #2287, .T. ) ;
#64340=ORIENTED_EDGE ( 'NONE', *, *, #28607, .T. ) ;
#64341=EDGE_CURVE ( 'NONE', #120440, #8844, #44159, .T. ) ;
#64342=PLANE ( 'NONE',  #4702 ) ;
#64343=DIRECTION ( 'NONE',  ( -0.000000000000000000, 1.000000000000000000, -0.000000000000000000 ) ) ;
#64344=EDGE_CURVE ( 'NONE', #107746, #49994, #35757, .T. ) ;
#64346=CARTESIAN_POINT ( 'NONE',  ( -7.700000000000012612, 2.500000000000000000, 4.776537180435972196 ) ) ;
#64347=CARTESIAN_POINT ( 'NONE',  ( -8.350000000000008527, 12.50000000000000000, 7.188010851410848723 ) ) ;
#64348=DIRECTION ( 'NONE',  ( 0.000000000000000000, 0.000000000000000000, 1.000000000000000000 ) ) ;
#64349=CARTESIAN_POINT ( 'NONE',  ( -5.000000000000026645, 2.500000000000000000, -3.537306695894649966 ) ) ;
#64350=VERTEX_POINT ( 'NONE', #68814 ) ;
#64351=DIRECTION ( 'NONE',  ( 0.000000000000000000, 0.000000000000000000, 1.000000000000000000 ) ) ;
#64352=AXIS2_PLACEMENT_3D ( 'NONE', #113286, #51172, #12509 ) ;
#64353=LINE ( 'NONE', #14593, #86053 ) ;
#64354=DIRECTION ( 'NONE',  ( 0.000000000000000000, 0.000000000000000000, 1.000000000000000000 ) ) ;
#64355=ORIENTED_EDGE ( 'NONE', *, *, #100123, .F. ) ;
#64356=CIRCLE ( 'NONE', #76891, 0.1000000000000000472 ) ;
#64357=DIRECTION ( 'NONE',  ( 0.000000000000000000, 0.000000000000000000, 1.000000000000000000 ) ) ;
#64358=AXIS2_PLACEMENT_3D ( 'NONE', #101493, #62220, #110654 ) ;
#64359=CIRCLE ( 'NONE', #7919, 0.1000000000000002554 ) ;
#64360=ORIENTED_EDGE ( 'NONE', *, *, #9385, .F. ) ;
#64361=DIRECTION ( 'NONE',  ( -0.000000000000000000, 1.000000000000000000, -0.000000000000000000 ) ) ;
#64362=ORIENTED_EDGE ( 'NONE', *, *, #77905, .F. ) ;
#64363=DIRECTION ( 'NONE',  ( 0.000000000000000000, 0.000000000000000000, -1.000000000000000000 ) ) ;
#64364=DIRECTION ( 'NONE',  ( 0.000000000000000000, 1.000000000000000000, 0.000000000000000000 ) ) ;
#64365=DIRECTION ( 'NONE',  ( 0.000000000000000000, 0.000000000000000000, 1.000000000000000000 ) ) ;
#64366=ORIENTED_EDGE ( 'NONE', *, *, #110666, .F. ) ;
#64367=AXIS2_PLACEMENT_3D ( 'NONE', #16405, #127676, #76651 ) ;
#64368=DIRECTION ( 'NONE',  ( 0.000000000000000000, -0.000000000000000000, 1.000000000000000000 ) ) ;
#64369=DIRECTION ( 'NONE',  ( 0.000000000000000000, 0.000000000000000000, 1.000000000000000000 ) ) ;
#64370=CONICAL_SURFACE ( 'NONE', #97819, 0.1000000000000002554, 0.003490658503988666988 ) ;
#64371=ADVANCED_FACE ( 'NONE', ( #19047 ), #59001, .T. ) ;
#64372=EDGE_LOOP ( 'NONE', ( #40966, #1461, #89694, #53644 ) ) ;
#64373=DIRECTION ( 'NONE',  ( -0.000000000000000000, 1.000000000000000000, -0.000000000000000000 ) ) ;
#64375=VECTOR ( 'NONE', #45719, 1000.000000000000000 ) ;
#64376=ORIENTED_EDGE ( 'NONE', *, *, #982, .T. ) ;
#64377=ADVANCED_FACE ( 'NONE', ( #53049 ), #117283, .T. ) ;
#64378=ORIENTED_EDGE ( 'NONE', *, *, #99197, .T. ) ;
#64379=FACE_OUTER_BOUND ( 'NONE', #18530, .T. ) ;
#64380=DIRECTION ( 'NONE',  ( 0.000000000000000000, 1.000000000000000000, 0.000000000000000000 ) ) ;
#64381=DIRECTION ( 'NONE',  ( 0.000000000000000000, 0.000000000000000000, -1.000000000000000000 ) ) ;
#64382=ORIENTED_EDGE ( 'NONE', *, *, #10432, .F. ) ;
#64383=AXIS2_PLACEMENT_3D ( 'NONE', #117375, #86657, #98398 ) ;
#64384=DIRECTION ( 'NONE',  ( 0.000000000000000000, 0.000000000000000000, 1.000000000000000000 ) ) ;
#64385=CARTESIAN_POINT ( 'NONE',  ( 6.899999999999928413, 2.500000000000000000, -4.776537180435977525 ) ) ;
#64386=AXIS2_PLACEMENT_3D ( 'NONE', #19702, #20345, #38726 ) ;
#64387=VERTEX_POINT ( 'NONE', #51763 ) ;
#64388=EDGE_CURVE ( 'NONE', #15926, #64820, #12745, .T. ) ;
#64389=CARTESIAN_POINT ( 'NONE',  ( 11.24999999999994493, 2.500000000000000000, 6.395190528383296602 ) ) ;
#64390=CARTESIAN_POINT ( 'NONE',  ( -2.499999999999996003, 2.500000000000000000, -4.330127018922201643 ) ) ;
#64391=AXIS2_PLACEMENT_3D ( 'NONE', #123914, #3511, #103646 ) ;
#64392=CARTESIAN_POINT ( 'NONE',  ( 15.39999999999989022, 2.500000000000000000, 0.09999999999999761857 ) ) ;
#64393=DIRECTION ( 'NONE',  ( 0.000000000000000000, 1.000000000000000000, 0.000000000000000000 ) ) ;
#64394=DIRECTION ( 'NONE',  ( -0.000000000000000000, 1.000000000000000000, -0.000000000000000000 ) ) ;
#64395=CARTESIAN_POINT ( 'NONE',  ( -10.85000000000000142, 12.50000000000000000, -6.495190528383298911 ) ) ;
#64396=CIRCLE ( 'NONE', #53940, 0.1000000000000002554 ) ;
#64397=DIRECTION ( 'NONE',  ( -0.000000000000000000, -1.000000000000000000, -0.000000000000000000 ) ) ;
#64398=ORIENTED_EDGE ( 'NONE', *, *, #109890, .T. ) ;
#64399=VERTEX_POINT ( 'NONE', #52395 ) ;
#64400=VERTEX_POINT ( 'NONE', #14387 ) ;
#64401=ORIENTED_EDGE ( 'NONE', *, *, #18790, .T. ) ;
#64402=DIRECTION ( 'NONE',  ( 0.000000000000000000, 0.000000000000000000, 1.000000000000000000 ) ) ;
#64403=DIRECTION ( 'NONE',  ( -0.000000000000000000, -1.000000000000000000, -0.000000000000000000 ) ) ;
#64404=PLANE ( 'NONE',  #73981 ) ;
#64405=CIRCLE ( 'NONE', #127122, 0.06509327318403745899 ) ;
#64406=VERTEX_POINT ( 'NONE', #32786 ) ;
#64407=FACE_BOUND ( 'NONE', #2176, .T. ) ;
#64408=EDGE_CURVE ( 'NONE', #9509, #18441, #16931, .T. ) ;
#64409=PLANE ( 'NONE',  #22869 ) ;
#64410=DIRECTION ( 'NONE',  ( 0.000000000000000000, 1.000000000000000000, 0.000000000000000000 ) ) ;
#64411=CARTESIAN_POINT ( 'NONE',  ( -8.749999999999971578, 2.500000000000000000, 6.495190528383297135 ) ) ;
#64412=AXIS2_PLACEMENT_3D ( 'NONE', #93769, #46591, #123855 ) ;
#64413=VECTOR ( 'NONE', #43935, 1000.000000000000000 ) ;
#64414=CARTESIAN_POINT ( 'NONE',  ( -8.550000000000011369, 2.500000000000000000, -2.511473670974877948 ) ) ;
#64415=FACE_OUTER_BOUND ( 'NONE', #83467, .T. ) ;
#64416=CARTESIAN_POINT ( 'NONE',  ( 4.149999999999938183, 2.500000000000000000, 5.902370205355745192 ) ) ;
#64417=LINE ( 'NONE', #125278, #32931 ) ;
#64418=DIRECTION ( 'NONE',  ( 0.000000000000000000, 0.000000000000000000, 1.000000000000000000 ) ) ;
#64419=CARTESIAN_POINT ( 'NONE',  ( 8.549999999999924327, 12.50000000000000000, -6.776507416713039689 ) ) ;
#64420=DIRECTION ( 'NONE',  ( 0.000000000000000000, 0.000000000000000000, -1.000000000000000000 ) ) ;
#64421=VERTEX_POINT ( 'NONE', #62866 ) ;
#64422=ORIENTED_EDGE ( 'NONE', *, *, #46584, .T. ) ;
#64423=ADVANCED_FACE ( 'NONE', ( #1355 ), #73972, .T. ) ;
#64424=ORIENTED_EDGE ( 'NONE', *, *, #62246, .T. ) ;
#64425=ORIENTED_EDGE ( 'NONE', *, *, #58168, .T. ) ;
#64426=CARTESIAN_POINT ( 'NONE',  ( -10.40000000000000213, 12.50000000000000000, 5.022947341949748790 ) ) ;
#64427=EDGE_LOOP ( 'NONE', ( #89754, #55386 ) ) ;
#64428=DIRECTION ( 'NONE',  ( 0.000000000000000000, 0.000000000000000000, 1.000000000000000000 ) ) ;
#64430=ORIENTED_EDGE ( 'NONE', *, *, #61874, .T. ) ;
#64431=DIRECTION ( 'NONE',  ( 0.000000000000000000, 0.000000000000000000, 1.000000000000000000 ) ) ;
#64432=CONICAL_SURFACE ( 'NONE', #60255, 0.09999999999999982514, 0.003490658503988666988 ) ;
#64433=CARTESIAN_POINT ( 'NONE',  ( 105.5000000000000142, -1.500000000000000222, -1.322875655532295136 ) ) ;
#64434=CARTESIAN_POINT ( 'NONE',  ( 8.149999999999923972, 2.500000000000000000, -6.841600689897077814 ) ) ;
#64435=CARTESIAN_POINT ( 'NONE',  ( -5.400000000000023448, 2.500000000000000000, -4.330127018922201643 ) ) ;
#64436=AXIS2_PLACEMENT_3D ( 'NONE', #114325, #15469, #16742 ) ;
#64437=ADVANCED_FACE ( 'NONE', ( #102769 ), #10686, .T. ) ;
#64438=EDGE_LOOP ( 'NONE', ( #117729, #79500, #110900, #99854 ) ) ;
#64439=CONICAL_SURFACE ( 'NONE', #70704, 0.1000000000000002554, 0.003490658503988666988 ) ;
#64440=EDGE_LOOP ( 'NONE', ( #97089, #33713 ) ) ;
#64441=CIRCLE ( 'NONE', #1735, 0.1000000000000002554 ) ;
#64442=EDGE_LOOP ( 'NONE', ( #69070, #71345, #39640, #1650 ) ) ;
#64443=DIRECTION ( 'NONE',  ( 0.000000000000000000, 1.000000000000000000, 0.000000000000000000 ) ) ;
#64444=EDGE_LOOP ( 'NONE', ( #99811, #98952, #67517, #107708 ) ) ;
#64445=DIRECTION ( 'NONE',  ( 0.05223670945016245515, 0.9986347311133432214, 0.000000000000000000 ) ) ;
#64446=ORIENTED_EDGE ( 'NONE', *, *, #86537, .F. ) ;
#64447=VERTEX_POINT ( 'NONE', #101506 ) ;
#64448=CONICAL_SURFACE ( 'NONE', #95854, 0.1000000000000002554, 0.003490658503988666988 ) ;
#64449=DIRECTION ( 'NONE',  ( -0.000000000000000000, -1.000000000000000000, -0.000000000000000000 ) ) ;
#64450=AXIS2_PLACEMENT_3D ( 'NONE', #60834, #12369, #1266 ) ;
#64451=DIRECTION ( 'NONE',  ( 0.000000000000000000, 0.000000000000000000, 1.000000000000000000 ) ) ;
#64452=DIRECTION ( 'NONE',  ( -0.000000000000000000, 1.000000000000000000, -0.000000000000000000 ) ) ;
#64453=CARTESIAN_POINT ( 'NONE',  ( -14.14999999999998792, 12.50000000000000000, -1.472243186433547901 ) ) ;
#64454=DIRECTION ( 'NONE',  ( -0.000000000000000000, -1.000000000000000000, -0.000000000000000000 ) ) ;
#64455=ORIENTED_EDGE ( 'NONE', *, *, #4285, .F. ) ;
#64456=DIRECTION ( 'NONE',  ( -0.000000000000000000, -1.000000000000000000, -0.000000000000000000 ) ) ;
#64457=CIRCLE ( 'NONE', #49818, 0.1000000000000002554 ) ;
#64458=ORIENTED_EDGE ( 'NONE', *, *, #89146, .T. ) ;
#64459=CARTESIAN_POINT ( 'NONE',  ( 87.50000000000002842, 5.708722954879577038, 4.899943752027911437 ) ) ;
#64460=ADVANCED_FACE ( 'NONE', ( #3300 ), #106839, .T. ) ;
#64461=ORIENTED_EDGE ( 'NONE', *, *, #3494, .T. ) ;
#64462=DIRECTION ( 'NONE',  ( 0.000000000000000000, -0.9999939076577903929, 0.003490651415223739937 ) ) ;
#64463=DIRECTION ( 'NONE',  ( 0.000000000000000000, 0.000000000000000000, -1.000000000000000000 ) ) ;
#64464=CONICAL_SURFACE ( 'NONE', #56048, 0.09999999999999982514, 0.003490658503988666988 ) ;
#64465=DIRECTION ( 'NONE',  ( 0.000000000000000000, 0.000000000000000000, 1.000000000000000000 ) ) ;
#64466=CARTESIAN_POINT ( 'NONE',  ( 12.49999999999990408, 12.50000000000000000, -3.637306695894650055 ) ) ;
#64467=ORIENTED_EDGE ( 'NONE', *, *, #20140, .F. ) ;
#64469=CARTESIAN_POINT ( 'NONE',  ( -11.24999999999996270, 12.50000000000000000, 2.230156782645134950 ) ) ;
#64470=CIRCLE ( 'NONE', #118853, 0.06509327318403745899 ) ;
#64472=CARTESIAN_POINT ( 'NONE',  ( 5.649999999999936406, 2.500000000000000000, -6.841600689897077814 ) ) ;
#64473=ORIENTED_EDGE ( 'NONE', *, *, #37481, .F. ) ;
#64474=ORIENTED_EDGE ( 'NONE', *, *, #42807, .T. ) ;
#64475=EDGE_CURVE ( 'NONE', #4913, #71367, #4417, .T. ) ;
#64476=EDGE_CURVE ( 'NONE', #4284, #98451, #29498, .T. ) ;
#64477=EDGE_LOOP ( 'NONE', ( #14042, #40479, #64864, #117600 ) ) ;
#64478=CARTESIAN_POINT ( 'NONE',  ( -13.54999999999998828, 12.50000000000000000, -2.576566944158912964 ) ) ;
#64479=CARTESIAN_POINT ( 'NONE',  ( 13.34999999999990017, 12.50000000000000000, 1.472243186433545459 ) ) ;
#64480=EDGE_CURVE ( 'NONE', #25579, #30916, #123564, .T. ) ;
#64482=EDGE_CURVE ( 'NONE', #21022, #125373, #127687, .T. ) ;
#64483=DIRECTION ( 'NONE',  ( 0.000000000000000000, 0.000000000000000000, -1.000000000000000000 ) ) ;
#64484=AXIS2_PLACEMENT_3D ( 'NONE', #27407, #99886, #107274 ) ;
#64485=FACE_OUTER_BOUND ( 'NONE', #12992, .T. ) ;
#64486=DIRECTION ( 'NONE',  ( -4.274815082592931898E-19, -0.9999939076577903929, -0.003490651415223739937 ) ) ;
#64487=EDGE_CURVE ( 'NONE', #17095, #111595, #102642, .T. ) ;
#64488=ADVANCED_FACE ( 'NONE', ( #3934 ), #125622, .T. ) ;
#64489=CIRCLE ( 'NONE', #41535, 0.1000000000000000472 ) ;
#64490=EDGE_CURVE ( 'NONE', #105036, #82187, #71249, .T. ) ;
#64491=EDGE_LOOP ( 'NONE', ( #35671, #46308, #39607, #82248 ) ) ;
#64492=EDGE_CURVE ( 'NONE', #14447, #61230, #100671, .T. ) ;
#64493=CARTESIAN_POINT ( 'NONE',  ( -5.850000000000019185, 2.500000000000000000, 2.165063509461097713 ) ) ;
#64494=EDGE_CURVE ( 'NONE', #1314, #124558, #56879, .T. ) ;
#64495=ORIENTED_EDGE ( 'NONE', *, *, #124330, .T. ) ;
#64496=AXIS2_PLACEMENT_3D ( 'NONE', #128000, #65846, #17378 ) ;
#64497=CARTESIAN_POINT ( 'NONE',  ( 1.449999999999952216, 12.50000000000000000, 1.818653347947321475 ) ) ;
#64498=CARTESIAN_POINT ( 'NONE',  ( 5.849999999999932143, 2.500000000000000000, 2.265063509461097357 ) ) ;
#64499=DIRECTION ( 'NONE',  ( -0.000000000000000000, 1.000000000000000000, -0.000000000000000000 ) ) ;
#64500=ADVANCED_FACE ( 'NONE', ( #35981 ), #73485, .T. ) ;
#64501=ORIENTED_EDGE ( 'NONE', *, *, #116613, .F. ) ;
#64502=VECTOR ( 'NONE', #127471, 1000.000000000000000 ) ;
#64503=CARTESIAN_POINT ( 'NONE',  ( -13.34999999999999076, 2.500000000000000000, -1.472243186433547901 ) ) ;
#64504=FACE_OUTER_BOUND ( 'NONE', #42367, .T. ) ;
#64505=VERTEX_POINT ( 'NONE', #55619 ) ;
#64506=CARTESIAN_POINT ( 'NONE',  ( 4.349999999999940137, 2.500000000000000000, -2.511473670974877948 ) ) ;
#64507=ORIENTED_EDGE ( 'NONE', *, *, #74846, .F. ) ;
#64508=VERTEX_POINT ( 'NONE', #84435 ) ;
#64509=CARTESIAN_POINT ( 'NONE',  ( -5.400000000000019895, 12.50000000000000000, 4.330127018922196314 ) ) ;
#64510=AXIS2_PLACEMENT_3D ( 'NONE', #61005, #100302, #30288 ) ;
#64511=ORIENTED_EDGE ( 'NONE', *, *, #53282, .F. ) ;
#64512=CARTESIAN_POINT ( 'NONE',  ( 16.72050902517006676, 2.552201582238759592, -5.918448581778455342 ) ) ;
#64513=DIRECTION ( 'NONE',  ( 0.000000000000000000, -0.000000000000000000, 1.000000000000000000 ) ) ;
#64514=DIRECTION ( 'NONE',  ( 0.000000000000000000, 0.000000000000000000, 1.000000000000000000 ) ) ;
#64516=AXIS2_PLACEMENT_3D ( 'NONE', #44539, #77224, #66747 ) ;
#64517=FACE_BOUND ( 'NONE', #90297, .T. ) ;
#64519=CIRCLE ( 'NONE', #62492, 0.06509327318403745899 ) ;
#64520=DIRECTION ( 'NONE',  ( 0.000000000000000000, 0.000000000000000000, -1.000000000000000000 ) ) ;
#64521=DIRECTION ( 'NONE',  ( 0.000000000000000000, 0.000000000000000000, 1.000000000000000000 ) ) ;
#64522=EDGE_LOOP ( 'NONE', ( #53698, #68672, #87889, #28336 ) ) ;
#64523=CARTESIAN_POINT ( 'NONE',  ( 0.6499999999999543920, 2.500000000000000000, 6.248780366869521430 ) ) ;
#64524=CARTESIAN_POINT ( 'NONE',  ( -6.850000000000017408, 12.50000000000000000, -2.511473670974877948 ) ) ;
#64525=EDGE_LOOP ( 'NONE', ( #40755, #39338 ) ) ;
#64527=ADVANCED_FACE ( 'NONE', ( #106649 ), #67333, .T. ) ;
#64528=CIRCLE ( 'NONE', #106388, 0.1000000000000002554 ) ;
#64529=ORIENTED_EDGE ( 'NONE', *, *, #102598, .F. ) ;
#64530=AXIS2_PLACEMENT_3D ( 'NONE', #21779, #61708, #30962 ) ;
#64531=ADVANCED_FACE ( 'NONE', ( #117095 ), #81799, .T. ) ;
#64532=ORIENTED_EDGE ( 'NONE', *, *, #29162, .F. ) ;
#64533=DIRECTION ( 'NONE',  ( -0.000000000000000000, 1.000000000000000000, -0.000000000000000000 ) ) ;
#64534=CARTESIAN_POINT ( 'NONE',  ( -5.650000000000019895, 2.500000000000000000, 6.941600689897073018 ) ) ;
#64535=CARTESIAN_POINT ( 'NONE',  ( -10.80000000000000071, 12.50000000000000000, -2.276824562219559311E-15 ) ) ;
#64536=FACE_BOUND ( 'NONE', #119010, .T. ) ;
#64537=ORIENTED_EDGE ( 'NONE', *, *, #25578, .T. ) ;
#64539=AXIS2_PLACEMENT_3D ( 'NONE', #97857, #89340, #129290 ) ;
#64540=FACE_OUTER_BOUND ( 'NONE', #84630, .T. ) ;
#64541=DIRECTION ( 'NONE',  ( 0.000000000000000000, 0.000000000000000000, 1.000000000000000000 ) ) ;
#64542=EDGE_CURVE ( 'NONE', #121499, #112116, #44239, .T. ) ;
#64543=AXIS2_PLACEMENT_3D ( 'NONE', #24246, #85090, #64160 ) ;
#64544=CARTESIAN_POINT ( 'NONE',  ( -6.249999999999984901, 2.500000000000000000, -6.495190528383302464 ) ) ;
#64546=CARTESIAN_POINT ( 'NONE',  ( 3.149999999999944400, 2.500000000000000000, 1.818653347947321475 ) ) ;
#64547=DIRECTION ( 'NONE',  ( 0.000000000000000000, 0.000000000000000000, 1.000000000000000000 ) ) ;
#64548=AXIS2_PLACEMENT_3D ( 'NONE', #21437, #100630, #1156 ) ;
#64549=CARTESIAN_POINT ( 'NONE',  ( -6.515322082341305988E-15, 12.50000000000000000, 4.265033745738159077 ) ) ;
#64550=ORIENTED_EDGE ( 'NONE', *, *, #581, .F. ) ;
#64551=VERTEX_POINT ( 'NONE', #85713 ) ;
#64552=ORIENTED_EDGE ( 'NONE', *, *, #122452, .F. ) ;
#64553=VERTEX_POINT ( 'NONE', #76551 ) ;
#64554=VERTEX_POINT ( 'NONE', #24873 ) ;
#64555=CIRCLE ( 'NONE', #95871, 0.06509327318403745899 ) ;
#64556=PLANE ( 'NONE',  #100732 ) ;
#64557=FACE_OUTER_BOUND ( 'NONE', #80897, .T. ) ;
#64558=ORIENTED_EDGE ( 'NONE', *, *, #121169, .F. ) ;
#64559=FACE_BOUND ( 'NONE', #65244, .T. ) ;
#64560=CARTESIAN_POINT ( 'NONE',  ( -2.050000000000032685, 2.500000000000000000, -6.495190528383302464 ) ) ;
#64561=AXIS2_PLACEMENT_3D ( 'NONE', #79613, #38421, #30538 ) ;
#64562=DIRECTION ( 'NONE',  ( 0.000000000000000000, 0.000000000000000000, 1.000000000000000000 ) ) ;
#64563=ORIENTED_EDGE ( 'NONE', *, *, #27275, .T. ) ;
#64565=DIRECTION ( 'NONE',  ( 0.000000000000000000, 0.000000000000000000, 1.000000000000000000 ) ) ;
#64566=CARTESIAN_POINT ( 'NONE',  ( 4.999999999999935163, 2.500000000000000000, 3.537306695894645081 ) ) ;
#64567=EDGE_LOOP ( 'NONE', ( #16486, #128133 ) ) ;
#64568=CONICAL_SURFACE ( 'NONE', #10202, 0.09999999999999982514, 0.003490658503988666988 ) ;
#64569=DIRECTION ( 'NONE',  ( -0.000000000000000000, 1.000000000000000000, -0.000000000000000000 ) ) ;
#64570=ADVANCED_FACE ( 'NONE', ( #17615 ), #37283, .T. ) ;
#64571=CIRCLE ( 'NONE', #81310, 0.06509327318403745899 ) ;
#64572=ORIENTED_EDGE ( 'NONE', *, *, #82978, .F. ) ;
#64573=ORIENTED_EDGE ( 'NONE', *, *, #108251, .F. ) ;
#64574=ORIENTED_EDGE ( 'NONE', *, *, #66721, .F. ) ;
#64575=CARTESIAN_POINT ( 'NONE',  ( -4.550000000000026468, 2.500000000000000000, -6.595190528383302109 ) ) ;
#64576=CARTESIAN_POINT ( 'NONE',  ( -9.400000000000007461, 2.500000000000000000, 0.2464101615137735679 ) ) ;
#64577=DIRECTION ( 'NONE',  ( 0.000000000000000000, 0.000000000000000000, -1.000000000000000000 ) ) ;
#64578=CONICAL_SURFACE ( 'NONE', #22841, 0.1000000000000000472, 0.003490658503988666988 ) ;
#64579=ORIENTED_EDGE ( 'NONE', *, *, #25162, .T. ) ;
#64580=DIRECTION ( 'NONE',  ( 0.000000000000000000, 0.000000000000000000, 1.000000000000000000 ) ) ;
#64581=DIRECTION ( 'NONE',  ( 0.000000000000000000, -0.000000000000000000, 1.000000000000000000 ) ) ;
#64582=CIRCLE ( 'NONE', #110837, 0.1000000000000002554 ) ;
#64583=FACE_OUTER_BOUND ( 'NONE', #42974, .T. ) ;
#64584=AXIS2_PLACEMENT_3D ( 'NONE', #11072, #92215, #39921 ) ;
#64586=DIRECTION ( 'NONE',  ( 0.000000000000000000, 1.000000000000000000, 0.000000000000000000 ) ) ;
#64588=ADVANCED_FACE ( 'NONE', ( #96821 ), #119454, .T. ) ;
#64589=AXIS2_PLACEMENT_3D ( 'NONE', #100471, #80844, #89995 ) ;
#64590=CARTESIAN_POINT ( 'NONE',  ( 13.54999999999990123, 2.500000000000000000, 1.718653347947321386 ) ) ;
#64592=ORIENTED_EDGE ( 'NONE', *, *, #21842, .F. ) ;
#64593=FACE_OUTER_BOUND ( 'NONE', #118006, .T. ) ;
#64594=AXIS2_PLACEMENT_3D ( 'NONE', #54805, #115009, #5065 ) ;
#64595=AXIS2_PLACEMENT_3D ( 'NONE', #69838, #110393, #28632 ) ;
#64596=ORIENTED_EDGE ( 'NONE', *, *, #1557, .F. ) ;
#64597=VERTEX_POINT ( 'NONE', #116460 ) ;
#64598=DIRECTION ( 'NONE',  ( -0.000000000000000000, 1.000000000000000000, -0.000000000000000000 ) ) ;
#64599=PLANE ( 'NONE',  #19528 ) ;
#64600=DIRECTION ( 'NONE',  ( 0.000000000000000000, 0.000000000000000000, 1.000000000000000000 ) ) ;
#64601=CARTESIAN_POINT ( 'NONE',  ( -7.900000000000014566, 2.500000000000000000, -2.276824562219559311E-15 ) ) ;
#64602=EDGE_CURVE ( 'NONE', #76320, #10651, #31648, .T. ) ;
#64603=CARTESIAN_POINT ( 'NONE',  ( 14.14999999999989200, 12.50000000000000000, -2.165063509461101710 ) ) ;
#64604=ORIENTED_EDGE ( 'NONE', *, *, #97778, .T. ) ;
#64605=EDGE_LOOP ( 'NONE', ( #104903, #82423 ) ) ;
#64606=CARTESIAN_POINT ( 'NONE',  ( -11.24999999999996447, 12.50000000000000000, -2.165063509461097713 ) ) ;
#64607=DIRECTION ( 'NONE',  ( -0.000000000000000000, 1.000000000000000000, -0.000000000000000000 ) ) ;
#64608=DIRECTION ( 'NONE',  ( -0.000000000000000000, 1.000000000000000000, -0.000000000000000000 ) ) ;
#64609=CONICAL_SURFACE ( 'NONE', #45746, 0.1000000000000002554, 0.003490658503988666988 ) ;
#64610=EDGE_LOOP ( 'NONE', ( #113383, #57615 ) ) ;
#64611=ORIENTED_EDGE ( 'NONE', *, *, #35914, .F. ) ;
#64612=CARTESIAN_POINT ( 'NONE',  ( 11.89999999999990443, 2.500000000000000000, -0.4464101615137782142 ) ) ;
#64613=ORIENTED_EDGE ( 'NONE', *, *, #20141, .T. ) ;
#64614=DIRECTION ( 'NONE',  ( -0.000000000000000000, -1.000000000000000000, -0.000000000000000000 ) ) ;
#64615=AXIS2_PLACEMENT_3D ( 'NONE', #104587, #94773, #14885 ) ;
#64616=CIRCLE ( 'NONE', #112752, 0.06509327318403745899 ) ;
#64617=DIRECTION ( 'NONE',  ( 0.000000000000000000, 0.000000000000000000, -1.000000000000000000 ) ) ;
#64618=ORIENTED_EDGE ( 'NONE', *, *, #115159, .F. ) ;
#64619=DIRECTION ( 'NONE',  ( 0.000000000000000000, -0.9999939076577903929, 0.003490651415223739937 ) ) ;
#64620=CARTESIAN_POINT ( 'NONE',  ( -11.64999999999999680, 12.50000000000000000, 2.165063509461097713 ) ) ;
#64621=DIRECTION ( 'NONE',  ( -0.000000000000000000, -1.000000000000000000, -0.000000000000000000 ) ) ;
#64622=DIRECTION ( 'NONE',  ( 0.000000000000000000, 1.000000000000000000, 0.000000000000000000 ) ) ;
#64623=VERTEX_POINT ( 'NONE', #5216 ) ;
#64624=AXIS2_PLACEMENT_3D ( 'NONE', #14221, #15514, #122915 ) ;
#64625=EDGE_CURVE ( 'NONE', #16131, #125502, #35849, .T. ) ;
#64626=AXIS2_PLACEMENT_3D ( 'NONE', #77321, #67473, #64914 ) ;
#64627=CARTESIAN_POINT ( 'NONE',  ( -0.8500000000000382805, 2.500000000000000000, -2.757883832488654097 ) ) ;
#64628=DIRECTION ( 'NONE',  ( 0.000000000000000000, 0.000000000000000000, 1.000000000000000000 ) ) ;
#64629=ORIENTED_EDGE ( 'NONE', *, *, #118872, .T. ) ;
#64630=EDGE_LOOP ( 'NONE', ( #23298, #22571, #126662, #75313 ) ) ;
#64631=EDGE_CURVE ( 'NONE', #72890, #80189, #95550, .T. ) ;
#64633=CARTESIAN_POINT ( 'NONE',  ( -12.49999999999999289, 2.500000000000000000, -0.6928203230275500335 ) ) ;
#64635=CIRCLE ( 'NONE', #16593, 0.06509327318403745899 ) ;
#64636=EDGE_CURVE ( 'NONE', #122361, #60183, #85995, .T. ) ;
#64637=DIRECTION ( 'NONE',  ( 0.000000000000000000, -0.9999939076577903929, 0.003490651415223739937 ) ) ;
#64638=LINE ( 'NONE', #104564, #94662 ) ;
#64639=AXIS2_PLACEMENT_3D ( 'NONE', #47443, #65287, #123561 ) ;
#64640=DIRECTION ( 'NONE',  ( 0.000000000000000000, 0.000000000000000000, -1.000000000000000000 ) ) ;
#64641=DIRECTION ( 'NONE',  ( -0.000000000000000000, -1.000000000000000000, -0.000000000000000000 ) ) ;
#64642=CARTESIAN_POINT ( 'NONE',  ( 0.1999999999999576006, 2.500000000000000000, -4.676537180435978769 ) ) ;
#64643=DIRECTION ( 'NONE',  ( 0.000000000000000000, -0.000000000000000000, 1.000000000000000000 ) ) ;
#64644=ADVANCED_FACE ( 'NONE', ( #56257 ), #21260, .T. ) ;
#64645=EDGE_CURVE ( 'NONE', #38017, #94907, #96175, .T. ) ;
#64647=DIRECTION ( 'NONE',  ( -0.000000000000000000, -1.000000000000000000, -0.000000000000000000 ) ) ;
#64648=VERTEX_POINT ( 'NONE', #66714 ) ;
#64649=ORIENTED_EDGE ( 'NONE', *, *, #60791, .F. ) ;
#64650=EDGE_CURVE ( 'NONE', #58293, #105467, #98518, .T. ) ;
#64651=ORIENTED_EDGE ( 'NONE', *, *, #103066, .F. ) ;
#64652=EDGE_LOOP ( 'NONE', ( #77788, #9757, #32149, #62854 ) ) ;
#64653=EDGE_CURVE ( 'NONE', #95822, #127721, #23307, .T. ) ;
#64654=CARTESIAN_POINT ( 'NONE',  ( 1.049999999999952971, 12.50000000000000000, 6.148780366869520897 ) ) ;
#64655=DIRECTION ( 'NONE',  ( 0.000000000000000000, 0.000000000000000000, 1.000000000000000000 ) ) ;
#64656=CARTESIAN_POINT ( 'NONE',  ( 12.49999999999993605, 12.50000000000000000, -2.276824562219559311E-15 ) ) ;
#64657=EDGE_CURVE ( 'NONE', #98934, #117161, #40055, .T. ) ;
#64658=EDGE_LOOP ( 'NONE', ( #40511, #50858, #70899, #32286 ) ) ;
#64659=DIRECTION ( 'NONE',  ( 0.000000000000000000, 0.000000000000000000, 1.000000000000000000 ) ) ;
#64660=FACE_OUTER_BOUND ( 'NONE', #113821, .T. ) ;
#64661=DIRECTION ( 'NONE',  ( 0.000000000000000000, -0.9999939076577903929, 0.003490651415223739937 ) ) ;
#64662=ORIENTED_EDGE ( 'NONE', *, *, #927, .T. ) ;
#64663=CARTESIAN_POINT ( 'NONE',  ( -13.09999999999999254, 2.500000000000000000, 0.4464101615137777701 ) ) ;
#64664=DIRECTION ( 'NONE',  ( 0.000000000000000000, 0.000000000000000000, -1.000000000000000000 ) ) ;
#64665=ORIENTED_EDGE ( 'NONE', *, *, #81198, .T. ) ;
#64666=VERTEX_POINT ( 'NONE', #69287 ) ;
#64667=VERTEX_POINT ( 'NONE', #39238 ) ;
#64669=CARTESIAN_POINT ( 'NONE',  ( -3.300000000000028244, 12.50000000000000000, 4.330127018922196314 ) ) ;
#64670=CIRCLE ( 'NONE', #45902, 0.06509327318403745899 ) ;
#64671=DIRECTION ( 'NONE',  ( 0.000000000000000000, -0.000000000000000000, 1.000000000000000000 ) ) ;
#64672=DIRECTION ( 'NONE',  ( 0.000000000000000000, 0.000000000000000000, 1.000000000000000000 ) ) ;
#64673=FACE_OUTER_BOUND ( 'NONE', #70488, .T. ) ;
#64674=VERTEX_POINT ( 'NONE', #89596 ) ;
#64675=AXIS2_PLACEMENT_3D ( 'NONE', #69818, #109745, #70459 ) ;
#64676=VECTOR ( 'NONE', #107849, 1000.000000000000000 ) ;
#64677=FACE_OUTER_BOUND ( 'NONE', #119577, .T. ) ;
#64678=ORIENTED_EDGE ( 'NONE', *, *, #38366, .T. ) ;
#64679=PLANE ( 'NONE',  #47557 ) ;
#64680=FACE_OUTER_BOUND ( 'NONE', #76700, .T. ) ;
#64681=CIRCLE ( 'NONE', #8242, 0.06509327318403745899 ) ;
#64682=DIRECTION ( 'NONE',  ( -0.000000000000000000, -1.000000000000000000, -0.000000000000000000 ) ) ;
#64683=CARTESIAN_POINT ( 'NONE',  ( 15.44463772192101914, -2.469073678227480695, 4.264595835263015111 ) ) ;
#64684=ORIENTED_EDGE ( 'NONE', *, *, #13373, .T. ) ;
#64685=CIRCLE ( 'NONE', #20784, 0.06509327318403745899 ) ;
#64686=AXIS2_PLACEMENT_3D ( 'NONE', #32198, #80640, #62920 ) ;
#64687=EDGE_CURVE ( 'NONE', #17776, #88360, #106931, .T. ) ;
#64688=VERTEX_POINT ( 'NONE', #119058 ) ;
#64689=EDGE_CURVE ( 'NONE', #91598, #89245, #113193, .T. ) ;
#64690=ORIENTED_EDGE ( 'NONE', *, *, #78371, .T. ) ;
#64691=CARTESIAN_POINT ( 'NONE',  ( 0.4499999999999569344, 2.500000000000000000, 2.165063509461097713 ) ) ;
#64692=CARTESIAN_POINT ( 'NONE',  ( -0.6500000000000398792, 12.50000000000000000, -6.841600689897078702 ) ) ;
#64693=DIRECTION ( 'NONE',  ( -4.274815082592931898E-19, -0.9999939076577903929, -0.003490651415223739937 ) ) ;
#64694=FACE_BOUND ( 'NONE', #44858, .T. ) ;
#64695=CARTESIAN_POINT ( 'NONE',  ( 4.199999999999939782, 2.500000000000000000, -0.1000000000000022815 ) ) ;
#64696=DIRECTION ( 'NONE',  ( -0.000000000000000000, -1.000000000000000000, -0.000000000000000000 ) ) ;
#64697=CARTESIAN_POINT ( 'NONE',  ( -7.500000000000015099, 2.500000000000000000, -0.6928203230275541413 ) ) ;
#64698=AXIS2_PLACEMENT_3D ( 'NONE', #27697, #48008, #88556 ) ;
#64700=FACE_OUTER_BOUND ( 'NONE', #3148, .T. ) ;
#64701=LINE ( 'NONE', #6396, #97208 ) ;
#64702=VERTEX_POINT ( 'NONE', #30694 ) ;
#64703=AXIS2_PLACEMENT_3D ( 'NONE', #41290, #121119, #30832 ) ;
#64704=AXIS2_PLACEMENT_3D ( 'NONE', #54194, #5074, #83655 ) ;
#64705=DIRECTION ( 'NONE',  ( 0.000000000000000000, 1.000000000000000000, 0.000000000000000000 ) ) ;
#64706=ORIENTED_EDGE ( 'NONE', *, *, #59932, .F. ) ;
#64707=ORIENTED_EDGE ( 'NONE', *, *, #30128, .T. ) ;
#64708=ORIENTED_EDGE ( 'NONE', *, *, #27303, .T. ) ;
#64709=VERTEX_POINT ( 'NONE', #20213 ) ;
#64710=DIRECTION ( 'NONE',  ( 0.000000000000000000, 0.000000000000000000, 1.000000000000000000 ) ) ;
#64711=FACE_BOUND ( 'NONE', #86444, .T. ) ;
#64712=LINE ( 'NONE', #104634, #26486 ) ;
#64713=AXIS2_PLACEMENT_3D ( 'NONE', #74807, #89131, #30877 ) ;
#64714=AXIS2_PLACEMENT_3D ( 'NONE', #12137, #59993, #11508 ) ;
#64715=CIRCLE ( 'NONE', #123299, 0.06509327318403745899 ) ;
#64716=AXIS2_PLACEMENT_3D ( 'NONE', #35325, #6454, #96792 ) ;
#64717=EDGE_LOOP ( 'NONE', ( #66882, #22274, #79428, #101386 ) ) ;
#64718=CARTESIAN_POINT ( 'NONE',  ( 48.67919755204864174, 3.179368040564874764, 5.083101272004578064 ) ) ;
#64719=PLANE ( 'NONE',  #87584 ) ;
#64720=AXIS2_PLACEMENT_3D ( 'NONE', #9328, #111378, #59085 ) ;
#64721=EDGE_LOOP ( 'NONE', ( #12892, #39188 ) ) ;
#64722=DIRECTION ( 'NONE',  ( 0.000000000000000000, 0.000000000000000000, -1.000000000000000000 ) ) ;
#64723=CARTESIAN_POINT ( 'NONE',  ( 9.999999999999948486, 2.500000000000000000, -4.330127018922201643 ) ) ;
#64724=CIRCLE ( 'NONE', #48024, 0.06509327318403745899 ) ;
#64725=ADVANCED_FACE ( 'NONE', ( #68012 ), #10770, .T. ) ;
#64726=AXIS2_PLACEMENT_3D ( 'NONE', #47312, #36855, #28969 ) ;
#64727=EDGE_LOOP ( 'NONE', ( #9114, #81797 ) ) ;
#64728=CARTESIAN_POINT ( 'NONE',  ( 6.649999999999930189, 12.50000000000000000, -1.472243186433550122 ) ) ;
#64729=CARTESIAN_POINT ( 'NONE',  ( -13.34999999999999076, 2.500000000000000000, -1.472243186433547901 ) ) ;
#64730=VECTOR ( 'NONE', #3981, 1000.000000000000000 ) ;
#64731=EDGE_CURVE ( 'NONE', #102116, #89245, #49045, .T. ) ;
#64732=ORIENTED_EDGE ( 'NONE', *, *, #88062, .F. ) ;
#64733=DIRECTION ( 'NONE',  ( 0.000000000000000000, 0.000000000000000000, 1.000000000000000000 ) ) ;
#64734=DIRECTION ( 'NONE',  ( 0.000000000000000000, -0.9999939076577903929, 0.003490651415223739937 ) ) ;
#64735=CARTESIAN_POINT ( 'NONE',  ( 3.349999999999944578, 2.500000000000000000, -1.472243186433550122 ) ) ;
#64737=VERTEX_POINT ( 'NONE', #552 ) ;
#64738=EDGE_CURVE ( 'NONE', #108389, #122356, #123649, .T. ) ;
#64739=ORIENTED_EDGE ( 'NONE', *, *, #125232, .F. ) ;
#64740=ADVANCED_FACE ( 'NONE', ( #10385 ), #8632, .T. ) ;
#64741=CARTESIAN_POINT ( 'NONE',  ( 14.99999999999992895, 12.50000000000000000, -2.276824562219559311E-15 ) ) ;
#64742=VERTEX_POINT ( 'NONE', #40517 ) ;
#64743=CARTESIAN_POINT ( 'NONE',  ( -8.100000000000010303, 2.500000000000000000, 4.776537180435972196 ) ) ;
#64744=DIRECTION ( 'NONE',  ( 0.000000000000000000, 0.000000000000000000, 1.000000000000000000 ) ) ;
#64745=EDGE_LOOP ( 'NONE', ( #16289, #116109, #89814, #128929 ) ) ;
#64746=EDGE_CURVE ( 'NONE', #96017, #45268, #70600, .T. ) ;
#64747=DIRECTION ( 'NONE',  ( 0.000000000000000000, 0.000000000000000000, -1.000000000000000000 ) ) ;
#64748=CARTESIAN_POINT ( 'NONE',  ( 4.349999999999937472, 2.500000000000000000, 6.941600689897073018 ) ) ;
#64750=CARTESIAN_POINT ( 'NONE',  ( 4.199999999999938005, 2.500000000000000000, 4.430127018922196847 ) ) ;
#64752=PLANE ( 'NONE',  #91264 ) ;
#64753=EDGE_LOOP ( 'NONE', ( #52259, #74751 ) ) ;
#64754=ORIENTED_EDGE ( 'NONE', *, *, #20516, .T. ) ;
#64755=FACE_OUTER_BOUND ( 'NONE', #65713, .T. ) ;
#64756=CARTESIAN_POINT ( 'NONE',  ( 1.899999999999951283, 2.500000000000000000, -4.576537180435977348 ) ) ;
#64757=CARTESIAN_POINT ( 'NONE',  ( 1.449999999999949551, 2.500000000000000000, 6.941600689897073018 ) ) ;
#64758=EDGE_LOOP ( 'NONE', ( #24667, #127296, #76981, #30482 ) ) ;
#64759=ORIENTED_EDGE ( 'NONE', *, *, #80, .T. ) ;
#64760=ORIENTED_EDGE ( 'NONE', *, *, #1233, .T. ) ;
#64761=CIRCLE ( 'NONE', #119144, 0.06509327318403745899 ) ;
#64762=FACE_OUTER_BOUND ( 'NONE', #34526, .T. ) ;
#64763=DIRECTION ( 'NONE',  ( 0.000000000000000000, 1.000000000000000000, 0.000000000000000000 ) ) ;
#64764=DIRECTION ( 'NONE',  ( 0.000000000000000000, 1.000000000000000000, 0.000000000000000000 ) ) ;
#64766=CIRCLE ( 'NONE', #112898, 0.06509327318403745899 ) ;
#64767=CONICAL_SURFACE ( 'NONE', #8328, 0.09999999999999982514, 0.003490658503988666988 ) ;
#64768=DIRECTION ( 'NONE',  ( -4.274815082592931898E-19, -0.9999939076577903929, -0.003490651415223739937 ) ) ;
#64770=CARTESIAN_POINT ( 'NONE',  ( -4.150000000000024336, 2.500000000000000000, -2.857883832488653741 ) ) ;
#64771=DIRECTION ( 'NONE',  ( 0.000000000000000000, 0.000000000000000000, 1.000000000000000000 ) ) ;
#64772=DIRECTION ( 'NONE',  ( 0.000000000000000000, -0.000000000000000000, 1.000000000000000000 ) ) ;
#64773=DIRECTION ( 'NONE',  ( -0.000000000000000000, 1.000000000000000000, -0.000000000000000000 ) ) ;
#64774=CIRCLE ( 'NONE', #71048, 0.1000000000000002554 ) ;
#64775=CIRCLE ( 'NONE', #16727, 0.1000000000000002554 ) ;
#64776=ORIENTED_EDGE ( 'NONE', *, *, #95842, .T. ) ;
#64777=ADVANCED_FACE ( 'NONE', ( #58844 ), #83950, .T. ) ;
#64778=LINE ( 'NONE', #104071, #4716 ) ;
#64779=VERTEX_POINT ( 'NONE', #128247 ) ;
#64780=ORIENTED_EDGE ( 'NONE', *, *, #11322, .F. ) ;
#64781=EDGE_CURVE ( 'NONE', #47940, #120491, #37899, .T. ) ;
#64782=DIRECTION ( 'NONE',  ( 0.000000000000000000, 0.000000000000000000, 1.000000000000000000 ) ) ;
#64783=DIRECTION ( 'NONE',  ( 0.000000000000000000, -0.9999939076577903929, 0.003490651415223739937 ) ) ;
#64784=DIRECTION ( 'NONE',  ( 0.000000000000000000, 0.000000000000000000, 1.000000000000000000 ) ) ;
#64785=EDGE_CURVE ( 'NONE', #91012, #331, #67196, .T. ) ;
#64786=CARTESIAN_POINT ( 'NONE',  ( 10.64999999999990976, 2.500000000000000000, 1.818653347947321475 ) ) ;
#64787=DIRECTION ( 'NONE',  ( -4.274815082592931898E-19, -0.9999939076577903929, -0.003490651415223739937 ) ) ;
#64788=DIRECTION ( 'NONE',  ( 0.000000000000000000, 0.000000000000000000, 1.000000000000000000 ) ) ;
#64789=FACE_OUTER_BOUND ( 'NONE', #85264, .T. ) ;
#64790=ORIENTED_EDGE ( 'NONE', *, *, #45262, .F. ) ;
#64792=EDGE_CURVE ( 'NONE', #50211, #45883, #111032, .T. ) ;
#64793=EDGE_CURVE ( 'NONE', #58087, #85979, #88043, .T. ) ;
#64794=EDGE_CURVE ( 'NONE', #116290, #18103, #98753, .T. ) ;
#64795=EDGE_CURVE ( 'NONE', #115059, #68377, #69439, .T. ) ;
#64796=DIRECTION ( 'NONE',  ( 0.000000000000000000, 0.000000000000000000, 1.000000000000000000 ) ) ;
#64797=ORIENTED_EDGE ( 'NONE', *, *, #118708, .T. ) ;
#64798=CIRCLE ( 'NONE', #75176, 0.09999999999999982514 ) ;
#64799=AXIS2_PLACEMENT_3D ( 'NONE', #66983, #107576, #98378 ) ;
#64801=EDGE_CURVE ( 'NONE', #41131, #111968, #81072, .T. ) ;
#64802=ORIENTED_EDGE ( 'NONE', *, *, #107319, .T. ) ;
#64803=ORIENTED_EDGE ( 'NONE', *, *, #79962, .F. ) ;
#64804=CARTESIAN_POINT ( 'NONE',  ( 15.19999999999989093, 12.50000000000000000, 0.4115034346978109769 ) ) ;
#64805=DIRECTION ( 'NONE',  ( -0.000000000000000000, 1.000000000000000000, -0.000000000000000000 ) ) ;
#64806=AXIS2_PLACEMENT_3D ( 'NONE', #21538, #91565, #11052 ) ;
#64807=EDGE_CURVE ( 'NONE', #71888, #120246, #6713, .T. ) ;
#64808=EDGE_CURVE ( 'NONE', #3359, #9476, #128033, .T. ) ;
#64809=DIRECTION ( 'NONE',  ( 0.000000000000000000, 0.000000000000000000, -1.000000000000000000 ) ) ;
#64810=CARTESIAN_POINT ( 'NONE',  ( -1.850000000000033840, 2.500000000000000000, 1.818653347947321475 ) ) ;
#64811=FACE_OUTER_BOUND ( 'NONE', #84650, .T. ) ;
#64812=ORIENTED_EDGE ( 'NONE', *, *, #40080, .F. ) ;
#64813=CARTESIAN_POINT ( 'NONE',  ( -10.65000000000000391, 2.500000000000000000, -1.818653347947322141 ) ) ;
#64814=CARTESIAN_POINT ( 'NONE',  ( 9.149999999999920419, 12.50000000000000000, -5.867463478539787225 ) ) ;
#64815=FACE_OUTER_BOUND ( 'NONE', #63407, .T. ) ;
#64816=CIRCLE ( 'NONE', #96117, 0.09999999999999982514 ) ;
#64817=ORIENTED_EDGE ( 'NONE', *, *, #50176, .F. ) ;
#64818=CIRCLE ( 'NONE', #25109, 0.06509327318403745899 ) ;
#64819=ORIENTED_EDGE ( 'NONE', *, *, #16877, .F. ) ;
#64820=VERTEX_POINT ( 'NONE', #63356 ) ;
#64821=DIRECTION ( 'NONE',  ( -0.000000000000000000, -1.000000000000000000, -0.000000000000000000 ) ) ;
#64822=AXIS2_PLACEMENT_3D ( 'NONE', #85123, #125057, #26219 ) ;
#64823=DIRECTION ( 'NONE',  ( 0.000000000000000000, 1.000000000000000000, 0.000000000000000000 ) ) ;
#64824=DIRECTION ( 'NONE',  ( -4.274815082592931898E-19, -0.9999939076577903929, -0.003490651415223739937 ) ) ;
#64825=CIRCLE ( 'NONE', #25120, 0.1000000000000000056 ) ;
#64826=ORIENTED_EDGE ( 'NONE', *, *, #78722, .T. ) ;
#64827=CARTESIAN_POINT ( 'NONE',  ( -10.60000000000000142, 2.500000000000000000, 4.776537180435972196 ) ) ;
#64828=CARTESIAN_POINT ( 'NONE',  ( 5.849999999999933031, 12.50000000000000000, -1.537336459617587581 ) ) ;
#64829=EDGE_CURVE ( 'NONE', #62883, #66532, #79914, .T. ) ;
#64830=CARTESIAN_POINT ( 'NONE',  ( 0.5999999999999547917, 12.50000000000000000, 3.918623584224382839 ) ) ;
#64831=CARTESIAN_POINT ( 'NONE',  ( 6.049999999999932321, 12.50000000000000000, -1.818653347947326138 ) ) ;
#64832=CARTESIAN_POINT ( 'NONE',  ( -4.350000000000023626, 2.500000000000000000, 1.818653347947321475 ) ) ;
#64833=VERTEX_POINT ( 'NONE', #62081 ) ;
#64834=DIRECTION ( 'NONE',  ( 0.000000000000000000, 1.000000000000000000, 0.000000000000000000 ) ) ;
#64835=EDGE_CURVE ( 'NONE', #117365, #72485, #71596, .T. ) ;
#64836=VERTEX_POINT ( 'NONE', #122289 ) ;
#64837=ORIENTED_EDGE ( 'NONE', *, *, #65031, .F. ) ;
#64838=DIRECTION ( 'NONE',  ( 0.000000000000000000, 0.000000000000000000, 1.000000000000000000 ) ) ;
#64839=FACE_BOUND ( 'NONE', #120996, .T. ) ;
#64840=CARTESIAN_POINT ( 'NONE',  ( -13.54999999999998828, 2.500000000000000000, 1.818653347947325472 ) ) ;
#64841=FACE_OUTER_BOUND ( 'NONE', #85838, .T. ) ;
#64842=DIRECTION ( 'NONE',  ( 0.000000000000000000, -0.000000000000000000, 1.000000000000000000 ) ) ;
#64843=EDGE_CURVE ( 'NONE', #94991, #6037, #15133, .T. ) ;
#64844=ORIENTED_EDGE ( 'NONE', *, *, #90348, .F. ) ;
#64845=VECTOR ( 'NONE', #107102, 1000.000000000000000 ) ;
#64846=ORIENTED_EDGE ( 'NONE', *, *, #10381, .F. ) ;
#64847=CARTESIAN_POINT ( 'NONE',  ( 6.049999999999935874, 2.500000000000000000, -6.741600689897077281 ) ) ;
#64848=CARTESIAN_POINT ( 'NONE',  ( -5.400000000000019895, 2.500000000000000000, 4.230127018922196669 ) ) ;
#64849=CARTESIAN_POINT ( 'NONE',  ( 4.599999999999938360, 2.500000000000000000, -0.5928203230275541635 ) ) ;
#64850=CARTESIAN_POINT ( 'NONE',  ( 13.54999999999989768, 2.500000000000000000, -2.511473670974877948 ) ) ;
#64851=ORIENTED_EDGE ( 'NONE', *, *, #110774, .T. ) ;
#64853=CIRCLE ( 'NONE', #127564, 0.1000000000000000056 ) ;
#64854=CIRCLE ( 'NONE', #25149, 0.06509327318403745899 ) ;
#64856=ORIENTED_EDGE ( 'NONE', *, *, #124648, .T. ) ;
#64857=CARTESIAN_POINT ( 'NONE',  ( -13.54999999999998828, 12.50000000000000000, 1.818653347947325472 ) ) ;
#64858=ORIENTED_EDGE ( 'NONE', *, *, #119965, .F. ) ;
#64859=FACE_BOUND ( 'NONE', #45914, .T. ) ;
#64860=FACE_OUTER_BOUND ( 'NONE', #36533, .T. ) ;
#64861=ORIENTED_EDGE ( 'NONE', *, *, #867, .T. ) ;
#64862=LINE ( 'NONE', #15094, #111230 ) ;
#64863=DIRECTION ( 'NONE',  ( 0.000000000000000000, -0.9999939076577903929, 0.003490651415223739937 ) ) ;
#64864=ORIENTED_EDGE ( 'NONE', *, *, #799, .T. ) ;
#64865=ORIENTED_EDGE ( 'NONE', *, *, #127445, .T. ) ;
#64867=DIRECTION ( 'NONE',  ( 0.000000000000000000, 0.000000000000000000, -1.000000000000000000 ) ) ;
#64868=CARTESIAN_POINT ( 'NONE',  ( 13.74999999999989342, 12.50000000000000000, -1.472243186433550122 ) ) ;
#64869=LINE ( 'NONE', #25587, #99637 ) ;
#64870=CARTESIAN_POINT ( 'NONE',  ( -5.600000000000020073, 2.500000000000000000, 4.676537180435972552 ) ) ;
#64871=PLANE ( 'NONE',  #64124 ) ;
#64873=AXIS2_PLACEMENT_3D ( 'NONE', #63495, #23562, #34699 ) ;
#64874=EDGE_CURVE ( 'NONE', #80227, #109551, #3790, .T. ) ;
#64875=AXIS2_PLACEMENT_3D ( 'NONE', #43083, #12289, #82994 ) ;
#64876=ORIENTED_EDGE ( 'NONE', *, *, #43106, .T. ) ;
#64877=ORIENTED_EDGE ( 'NONE', *, *, #91366, .F. ) ;
#64878=CARTESIAN_POINT ( 'NONE',  ( 8.949999999999915801, 2.500000000000000000, -1.818653347947326138 ) ) ;
#64879=LINE ( 'NONE', #34155, #126982 ) ;
#64880=DIRECTION ( 'NONE',  ( 0.000000000000000000, 0.000000000000000000, 1.000000000000000000 ) ) ;
#64881=CARTESIAN_POINT ( 'NONE',  ( 14.54999999999989591, 12.50000000000000000, 2.165063509461097713 ) ) ;
#64882=ORIENTED_EDGE ( 'NONE', *, *, #100325, .T. ) ;
#64883=VERTEX_POINT ( 'NONE', #113093 ) ;
#64884=EDGE_CURVE ( 'NONE', #27262, #80417, #33273, .T. ) ;
#64885=FACE_BOUND ( 'NONE', #44666, .T. ) ;
#64886=ORIENTED_EDGE ( 'NONE', *, *, #96394, .T. ) ;
#64887=EDGE_CURVE ( 'NONE', #14356, #73692, #27656, .T. ) ;
#64888=FACE_OUTER_BOUND ( 'NONE', #43030, .T. ) ;
#64889=DIRECTION ( 'NONE',  ( -0.000000000000000000, -1.000000000000000000, -0.000000000000000000 ) ) ;
#64890=AXIS2_PLACEMENT_3D ( 'NONE', #66607, #97999, #37172 ) ;
#64891=VERTEX_POINT ( 'NONE', #61442 ) ;
#64892=CARTESIAN_POINT ( 'NONE',  ( -10.45000000000000107, 12.50000000000000000, 2.165063509461097713 ) ) ;
#64893=FACE_OUTER_BOUND ( 'NONE', #82943, .T. ) ;
#64895=CARTESIAN_POINT ( 'NONE',  ( 3.549999999999944755, 2.500000000000000000, -2.411473670974877859 ) ) ;
#64896=EDGE_CURVE ( 'NONE', #17226, #39251, #123546, .T. ) ;
#64897=CARTESIAN_POINT ( 'NONE',  ( 8.749999999999918288, 12.50000000000000000, -1.472243186433550122 ) ) ;
#64898=DIRECTION ( 'NONE',  ( -0.000000000000000000, 1.000000000000000000, -0.000000000000000000 ) ) ;
#64899=CARTESIAN_POINT ( 'NONE',  ( -3.300000000000027800, 2.500000000000000000, -2.276824562219559311E-15 ) ) ;
#64900=DIRECTION ( 'NONE',  ( 0.000000000000000000, 0.000000000000000000, 1.000000000000000000 ) ) ;
#64901=ADVANCED_FACE ( 'NONE', ( #52893 ), #56903, .T. ) ;
#64902=FACE_OUTER_BOUND ( 'NONE', #126896, .T. ) ;
#64903=AXIS2_PLACEMENT_3D ( 'NONE', #39424, #51163, #58408 ) ;
#64904=VERTEX_POINT ( 'NONE', #31335 ) ;
#64905=VERTEX_POINT ( 'NONE', #121617 ) ;
#64906=CONICAL_SURFACE ( 'NONE', #87880, 0.09999999999999982514, 0.003490658503988666988 ) ;
#64907=ORIENTED_EDGE ( 'NONE', *, *, #32846, .F. ) ;
#64908=LINE ( 'NONE', #27548, #5298 ) ;
#64909=EDGE_LOOP ( 'NONE', ( #96370, #54818 ) ) ;
#64910=LINE ( 'NONE', #1006, #22695 ) ;
#64911=ORIENTED_EDGE ( 'NONE', *, *, #29954, .F. ) ;
#64912=ORIENTED_EDGE ( 'NONE', *, *, #51996, .F. ) ;
#64914=DIRECTION ( 'NONE',  ( 0.000000000000000000, 0.000000000000000000, 1.000000000000000000 ) ) ;
#64915=AXIS2_PLACEMENT_3D ( 'NONE', #39294, #79823, #29445 ) ;
#64916=CARTESIAN_POINT ( 'NONE',  ( -11.89999999999999680, 2.500000000000000000, -4.676537180435976104 ) ) ;
#64918=CARTESIAN_POINT ( 'NONE',  ( 43.31340625576489600, -2.029328411527076437, -5.113049425671298387 ) ) ;
#64919=CIRCLE ( 'NONE', #94171, 0.1000000000000002554 ) ;
#64920=DIRECTION ( 'NONE',  ( 0.000000000000000000, 0.000000000000000000, -1.000000000000000000 ) ) ;
#64921=CARTESIAN_POINT ( 'NONE',  ( -11.25000000000000000, 2.500000000000000000, -2.857883832488649745 ) ) ;
#64922=VERTEX_POINT ( 'NONE', #112468 ) ;
#64923=DIRECTION ( 'NONE',  ( 0.000000000000000000, 0.000000000000000000, -1.000000000000000000 ) ) ;
#64924=EDGE_LOOP ( 'NONE', ( #53988, #53907, #69953, #32467 ) ) ;
#64925=EDGE_LOOP ( 'NONE', ( #129563, #6172 ) ) ;
#64926=VERTEX_POINT ( 'NONE', #23417 ) ;
#64927=DIRECTION ( 'NONE',  ( 0.000000000000000000, 0.000000000000000000, 1.000000000000000000 ) ) ;
#64929=ORIENTED_EDGE ( 'NONE', *, *, #18938, .T. ) ;
#64930=ORIENTED_EDGE ( 'NONE', *, *, #85385, .T. ) ;
#64932=CARTESIAN_POINT ( 'NONE',  ( 6.849999999999930367, 2.500000000000000000, -6.741600689897078169 ) ) ;
#64933=DIRECTION ( 'NONE',  ( 0.000000000000000000, 1.000000000000000000, 0.000000000000000000 ) ) ;
#64934=LINE ( 'NONE', #55773, #365 ) ;
#64935=CARTESIAN_POINT ( 'NONE',  ( -10.00000000000000533, 12.50000000000000000, 0.6928203230275494784 ) ) ;
#64936=CIRCLE ( 'NONE', #58696, 0.1000000000000000472 ) ;
#64937=EDGE_CURVE ( 'NONE', #86749, #92915, #44406, .T. ) ;
#64938=CARTESIAN_POINT ( 'NONE',  ( -1.850000000000033840, 2.500000000000000000, 6.941600689897073018 ) ) ;
#64939=VERTEX_POINT ( 'NONE', #120988 ) ;
#64940=CONICAL_SURFACE ( 'NONE', #8493, 0.1000000000000002554, 0.003490658503988666988 ) ;
#64941=EDGE_CURVE ( 'NONE', #102506, #59130, #54854, .T. ) ;
#64942=CIRCLE ( 'NONE', #41977, 0.09999999999999982514 ) ;
#64943=EDGE_CURVE ( 'NONE', #45085, #33480, #121669, .T. ) ;
#64944=DIRECTION ( 'NONE',  ( 0.000000000000000000, 0.000000000000000000, 1.000000000000000000 ) ) ;
#64945=ORIENTED_EDGE ( 'NONE', *, *, #11975, .F. ) ;
#64946=DIRECTION ( 'NONE',  ( 0.000000000000000000, 0.000000000000000000, 1.000000000000000000 ) ) ;
#64947=AXIS2_PLACEMENT_3D ( 'NONE', #38118, #55819, #87200 ) ;
#64948=ORIENTED_EDGE ( 'NONE', *, *, #70364, .F. ) ;
#64949=DIRECTION ( 'NONE',  ( 0.000000000000000000, 0.000000000000000000, 1.000000000000000000 ) ) ;
#64950=ADVANCED_FACE ( 'NONE', ( #1209 ), #125865, .T. ) ;
#64951=EDGE_LOOP ( 'NONE', ( #57013, #78483, #101159, #72125 ) ) ;
#64952=CONICAL_SURFACE ( 'NONE', #54571, 0.09999999999999982514, 0.003490658503988666988 ) ;
#64953=ORIENTED_EDGE ( 'NONE', *, *, #117045, .F. ) ;
#64954=DIRECTION ( 'NONE',  ( 0.000000000000000000, -0.000000000000000000, 1.000000000000000000 ) ) ;
#64955=FACE_OUTER_BOUND ( 'NONE', #85402, .T. ) ;
#64956=EDGE_CURVE ( 'NONE', #124385, #40490, #117537, .T. ) ;
#64957=ADVANCED_FACE ( 'NONE', ( #2480 ), #469, .T. ) ;
#64958=LINE ( 'NONE', #75423, #38433 ) ;
#64959=FACE_OUTER_BOUND ( 'NONE', #90982, .T. ) ;
#64960=ORIENTED_EDGE ( 'NONE', *, *, #8325, .F. ) ;
#64961=CARTESIAN_POINT ( 'NONE',  ( -9.800000000000006040, 2.500000000000000000, -4.676537180435974328 ) ) ;
#64962=CARTESIAN_POINT ( 'NONE',  ( 2.500000000000002220, 0.5000000000000002220, -9.999999999999998224 ) ) ;
#64963=FACE_OUTER_BOUND ( 'NONE', #4561, .T. ) ;
#64964=DIRECTION ( 'NONE',  ( 0.000000000000000000, -0.9999939076577903929, 0.003490651415223739937 ) ) ;
#64965=EDGE_CURVE ( 'NONE', #14028, #107104, #107086, .T. ) ;
#64966=DIRECTION ( 'NONE',  ( 0.000000000000000000, 1.000000000000000000, 0.000000000000000000 ) ) ;
#64967=EDGE_LOOP ( 'NONE', ( #72702, #70287, #3530, #59994 ) ) ;
#64968=EDGE_LOOP ( 'NONE', ( #53917, #51008, #57279, #18437 ) ) ;
#64970=ORIENTED_EDGE ( 'NONE', *, *, #69506, .T. ) ;
#64971=CARTESIAN_POINT ( 'NONE',  ( 6.849999999999927702, 2.500000000000000000, 2.511473670974873507 ) ) ;
#64972=AXIS2_PLACEMENT_3D ( 'NONE', #81236, #84, #72703 ) ;
#64973=DIRECTION ( 'NONE',  ( -0.000000000000000000, 1.000000000000000000, -0.000000000000000000 ) ) ;
#64974=CIRCLE ( 'NONE', #75442, 0.06509327318403745899 ) ;
#64976=DIRECTION ( 'NONE',  ( 0.000000000000000000, 0.000000000000000000, -1.000000000000000000 ) ) ;
#64977=CARTESIAN_POINT ( 'NONE',  ( 11.89999999999990798, 12.50000000000000000, -3.983716857408426293 ) ) ;
#64978=FACE_OUTER_BOUND ( 'NONE', #51757, .T. ) ;
#64979=DIRECTION ( 'NONE',  ( 0.000000000000000000, -0.9999939076577903929, 0.003490651415223739937 ) ) ;
#64980=ORIENTED_EDGE ( 'NONE', *, *, #16257, .T. ) ;
#64981=CIRCLE ( 'NONE', #90106, 0.06509327318403745899 ) ;
#64982=FACE_OUTER_BOUND ( 'NONE', #85317, .T. ) ;
#64983=FACE_OUTER_BOUND ( 'NONE', #24952, .T. ) ;
#64984=ORIENTED_EDGE ( 'NONE', *, *, #106983, .F. ) ;
#64985=FACE_OUTER_BOUND ( 'NONE', #5619, .T. ) ;
#64986=AXIS2_PLACEMENT_3D ( 'NONE', #58886, #73214, #62757 ) ;
#64987=AXIS2_PLACEMENT_3D ( 'NONE', #52147, #2368, #52781 ) ;
#64988=ADVANCED_FACE ( 'NONE', ( #35199 ), #21417, .T. ) ;
#64989=ORIENTED_EDGE ( 'NONE', *, *, #33724, .T. ) ;
#64990=DIRECTION ( 'NONE',  ( -0.000000000000000000, -1.000000000000000000, -0.000000000000000000 ) ) ;
#64991=ORIENTED_EDGE ( 'NONE', *, *, #10660, .T. ) ;
#64992=CARTESIAN_POINT ( 'NONE',  ( -4.150000000000024336, 2.500000000000000000, 2.065063509461097624 ) ) ;
#64993=DIRECTION ( 'NONE',  ( -0.000000000000000000, -1.000000000000000000, -0.000000000000000000 ) ) ;
#64995=AXIS2_PLACEMENT_3D ( 'NONE', #26069, #44412, #56780 ) ;
#64996=VERTEX_POINT ( 'NONE', #115662 ) ;
#64997=DIRECTION ( 'NONE',  ( -0.000000000000000000, -1.000000000000000000, -0.000000000000000000 ) ) ;
#64998=DIRECTION ( 'NONE',  ( 0.000000000000000000, 1.000000000000000000, 0.000000000000000000 ) ) ;
#64999=AXIS2_PLACEMENT_3D ( 'NONE', #32398, #63107, #72303 ) ;
#65000=ORIENTED_EDGE ( 'NONE', *, *, #21037, .T. ) ;
#65001=PLANE ( 'NONE',  #28549 ) ;
#65002=VERTEX_POINT ( 'NONE', #65921 ) ;
#65003=VERTEX_POINT ( 'NONE', #5706 ) ;
#65004=DIRECTION ( 'NONE',  ( 0.000000000000000000, -0.000000000000000000, 1.000000000000000000 ) ) ;
#65005=LINE ( 'NONE', #65663, #41677 ) ;
#65006=ORIENTED_EDGE ( 'NONE', *, *, #37211, .F. ) ;
#65007=DIRECTION ( 'NONE',  ( -0.000000000000000000, 1.000000000000000000, -0.000000000000000000 ) ) ;
#65008=LINE ( 'NONE', #36231, #21367 ) ;
#65009=EDGE_LOOP ( 'NONE', ( #81546, #4011, #36181, #62247 ) ) ;
#65010=DIRECTION ( 'NONE',  ( 0.000000000000000000, 0.000000000000000000, 1.000000000000000000 ) ) ;
#65012=CIRCLE ( 'NONE', #50460, 0.06509327318403745899 ) ;
#65013=FACE_OUTER_BOUND ( 'NONE', #41719, .T. ) ;
#65014=DIRECTION ( 'NONE',  ( 0.000000000000000000, 0.000000000000000000, 1.000000000000000000 ) ) ;
#65015=AXIS2_PLACEMENT_3D ( 'NONE', #7315, #119217, #127119 ) ;
#65016=AXIS2_PLACEMENT_3D ( 'NONE', #37593, #108247, #106947 ) ;
#65017=FACE_OUTER_BOUND ( 'NONE', #112124, .T. ) ;
#65019=ADVANCED_FACE ( 'NONE', ( #14237 ), #115381, .T. ) ;
#65020=ADVANCED_FACE ( 'NONE', ( #16158 ), #103927, .T. ) ;
#65021=CIRCLE ( 'NONE', #14843, 0.09999999999999982514 ) ;
#65022=ORIENTED_EDGE ( 'NONE', *, *, #124663, .T. ) ;
#65023=VERTEX_POINT ( 'NONE', #114376 ) ;
#65024=ORIENTED_EDGE ( 'NONE', *, *, #3809, .T. ) ;
#65025=ORIENTED_EDGE ( 'NONE', *, *, #13371, .F. ) ;
#65027=DIRECTION ( 'NONE',  ( -4.274815082592931898E-19, -0.9999939076577903929, -0.003490651415223739937 ) ) ;
#65028=CIRCLE ( 'NONE', #35813, 2.000000000000000000 ) ;
#65029=DIRECTION ( 'NONE',  ( -4.274815082592931898E-19, -0.9999939076577903929, -0.003490651415223739937 ) ) ;
#65030=VERTEX_POINT ( 'NONE', #45660 ) ;
#65031=EDGE_CURVE ( 'NONE', #120113, #51434, #94570, .T. ) ;
#65032=FACE_BOUND ( 'NONE', #115837, .T. ) ;
#65033=EDGE_CURVE ( 'NONE', #103864, #35250, #73639, .T. ) ;
#65034=FACE_OUTER_BOUND ( 'NONE', #111113, .T. ) ;
#65035=DIRECTION ( 'NONE',  ( 0.000000000000000000, 0.000000000000000000, 1.000000000000000000 ) ) ;
#65036=PLANE ( 'NONE',  #67927 ) ;
#65037=DIRECTION ( 'NONE',  ( 0.000000000000000000, 1.000000000000000000, 0.000000000000000000 ) ) ;
#65038=PLANE ( 'NONE',  #80537 ) ;
#65039=ADVANCED_FACE ( 'NONE', ( #66561 ), #55473, .T. ) ;
#65040=FACE_OUTER_BOUND ( 'NONE', #59898, .T. ) ;
#65041=EDGE_CURVE ( 'NONE', #124608, #46240, #31893, .T. ) ;
#65042=CARTESIAN_POINT ( 'NONE',  ( -11.84999999999999787, 2.500000000000000000, -6.841600689897074261 ) ) ;
#65043=CARTESIAN_POINT ( 'NONE',  ( 3.749999999999942268, 12.50000000000000000, -1.407149913249512663 ) ) ;
#65044=EDGE_CURVE ( 'NONE', #28259, #46373, #17179, .T. ) ;
#65045=DIRECTION ( 'NONE',  ( 0.000000000000000000, 0.000000000000000000, 1.000000000000000000 ) ) ;
#65046=ADVANCED_FACE ( 'NONE', ( #26658 ), #75692, .T. ) ;
#65047=ADVANCED_FACE ( 'NONE', ( #94103 ), #38147, .T. ) ;
#65048=DIRECTION ( 'NONE',  ( 0.000000000000000000, 0.000000000000000000, 1.000000000000000000 ) ) ;
#65049=ORIENTED_EDGE ( 'NONE', *, *, #114417, .F. ) ;
#65050=ORIENTED_EDGE ( 'NONE', *, *, #98337, .F. ) ;
#65051=ORIENTED_EDGE ( 'NONE', *, *, #32295, .T. ) ;
#65052=EDGE_LOOP ( 'NONE', ( #17328, #33323, #114125, #14162 ) ) ;
#65053=DIRECTION ( 'NONE',  ( 0.000000000000000000, 0.000000000000000000, 1.000000000000000000 ) ) ;
#65054=ORIENTED_EDGE ( 'NONE', *, *, #85283, .F. ) ;
#65055=CARTESIAN_POINT ( 'NONE',  ( -3.950000000000028155, 12.50000000000000000, -6.841600689897077814 ) ) ;
#65056=ORIENTED_EDGE ( 'NONE', *, *, #93158, .F. ) ;
#65057=EDGE_CURVE ( 'NONE', #112512, #97470, #86191, .T. ) ;
#65059=DIRECTION ( 'NONE',  ( 0.000000000000000000, 0.000000000000000000, 1.000000000000000000 ) ) ;
#65060=AXIS2_PLACEMENT_3D ( 'NONE', #13110, #53064, #23592 ) ;
#65061=CIRCLE ( 'NONE', #75530, 0.1000000000000002554 ) ;
#65062=DIRECTION ( 'NONE',  ( 0.000000000000000000, 0.000000000000000000, 1.000000000000000000 ) ) ;
#65063=DIRECTION ( 'NONE',  ( -4.274815082592931898E-19, -0.9999939076577903929, -0.003490651415223739937 ) ) ;
#65064=DIRECTION ( 'NONE',  ( 0.000000000000000000, 0.000000000000000000, 1.000000000000000000 ) ) ;
#65065=CARTESIAN_POINT ( 'NONE',  ( -11.24999999999996447, 12.50000000000000000, -6.430097255199260786 ) ) ;
#65066=ORIENTED_EDGE ( 'NONE', *, *, #13359, .T. ) ;
#65067=CONICAL_SURFACE ( 'NONE', #12744, 0.1000000000000002554, 0.003490658503988666988 ) ;
#65068=AXIS2_PLACEMENT_3D ( 'NONE', #64786, #94250, #86354 ) ;
#65069=ORIENTED_EDGE ( 'NONE', *, *, #14254, .T. ) ;
#65070=EDGE_LOOP ( 'NONE', ( #6144, #87032, #58163, #33549 ) ) ;
#65071=DIRECTION ( 'NONE',  ( -0.000000000000000000, -1.000000000000000000, -0.000000000000000000 ) ) ;
#65072=ORIENTED_EDGE ( 'NONE', *, *, #46925, .F. ) ;
#65073=DIRECTION ( 'NONE',  ( 0.000000000000000000, 0.000000000000000000, 1.000000000000000000 ) ) ;
#65075=ORIENTED_EDGE ( 'NONE', *, *, #8066, .T. ) ;
#65076=VERTEX_POINT ( 'NONE', #86854 ) ;
#65077=VECTOR ( 'NONE', #44390, 1000.000000000000000 ) ;
#65078=FACE_OUTER_BOUND ( 'NONE', #81454, .T. ) ;
#65079=AXIS2_PLACEMENT_3D ( 'NONE', #16699, #76294, #116203 ) ;
#65080=CARTESIAN_POINT ( 'NONE',  ( -8.150000000000009237, 12.50000000000000000, 6.841600689897072485 ) ) ;
#65082=CARTESIAN_POINT ( 'NONE',  ( -0.6500000000000403233, 2.500000000000000000, 1.818653347947321475 ) ) ;
#65083=AXIS2_PLACEMENT_3D ( 'NONE', #102504, #11538, #61944 ) ;
#65084=DIRECTION ( 'NONE',  ( -0.000000000000000000, 1.000000000000000000, -0.000000000000000000 ) ) ;
#65085=EDGE_CURVE ( 'NONE', #88607, #106514, #109138, .T. ) ;
#65086=CONICAL_SURFACE ( 'NONE', #104792, 0.1000000000000000472, 0.003490658503988666988 ) ;
#65087=VERTEX_POINT ( 'NONE', #84275 ) ;
#65088=EDGE_CURVE ( 'NONE', #46379, #69366, #34563, .T. ) ;
#65089=DIRECTION ( 'NONE',  ( -0.000000000000000000, -1.000000000000000000, -0.000000000000000000 ) ) ;
#65090=ORIENTED_EDGE ( 'NONE', *, *, #48109, .F. ) ;
#65091=CARTESIAN_POINT ( 'NONE',  ( 2.899999999999945732, 2.500000000000000000, -4.430127018922202176 ) ) ;
#65092=EDGE_CURVE ( 'NONE', #11512, #107667, #64638, .T. ) ;
#65093=VERTEX_POINT ( 'NONE', #94738 ) ;
#65094=FACE_OUTER_BOUND ( 'NONE', #73151, .T. ) ;
#65095=VECTOR ( 'NONE', #56082, 1000.000000000000000 ) ;
#65096=DIRECTION ( 'NONE',  ( 0.000000000000000000, -0.000000000000000000, 1.000000000000000000 ) ) ;
#65097=CARTESIAN_POINT ( 'NONE',  ( -8.550000000000013145, 2.500000000000000000, -6.841600689897073373 ) ) ;
#65098=EDGE_CURVE ( 'NONE', #60150, #97364, #48721, .T. ) ;
#65099=CARTESIAN_POINT ( 'NONE',  ( 4.999999999999935163, 2.500000000000000000, 0.6928203230275494784 ) ) ;
#65100=EDGE_LOOP ( 'NONE', ( #119220, #57955, #114407, #128121 ) ) ;
#65101=EDGE_CURVE ( 'NONE', #84066, #99278, #100915, .T. ) ;
#65102=DIRECTION ( 'NONE',  ( -0.000000000000000000, -1.000000000000000000, -0.000000000000000000 ) ) ;
#65103=ADVANCED_FACE ( 'NONE', ( #118898 ), #27766, .T. ) ;
#65104=ADVANCED_FACE ( 'NONE', ( #39077 ), #90446, .T. ) ;
#65105=DIRECTION ( 'NONE',  ( 0.000000000000000000, -0.000000000000000000, 1.000000000000000000 ) ) ;
#65106=ORIENTED_EDGE ( 'NONE', *, *, #9825, .F. ) ;
#65107=ORIENTED_EDGE ( 'NONE', *, *, #70254, .T. ) ;
#65108=ORIENTED_EDGE ( 'NONE', *, *, #59030, .T. ) ;
#65109=DIRECTION ( 'NONE',  ( 0.000000000000000000, 1.000000000000000000, 0.000000000000000000 ) ) ;
#65110=DIRECTION ( 'NONE',  ( 0.000000000000000000, 1.000000000000000000, 0.000000000000000000 ) ) ;
#65112=DIRECTION ( 'NONE',  ( 0.000000000000000000, 0.000000000000000000, -1.000000000000000000 ) ) ;
#65113=ADVANCED_FACE ( 'NONE', ( #28592 ), #88794, .T. ) ;
#65114=FACE_OUTER_BOUND ( 'NONE', #11969, .T. ) ;
#65115=DIRECTION ( 'NONE',  ( -0.000000000000000000, 1.000000000000000000, -0.000000000000000000 ) ) ;
#65116=CIRCLE ( 'NONE', #127821, 0.1000000000000002554 ) ;
#65117=AXIS2_PLACEMENT_3D ( 'NONE', #96040, #5072, #6336 ) ;
#65118=CONICAL_SURFACE ( 'NONE', #102775, 0.1000000000000002554, 0.003490658503988666988 ) ;
#65119=ORIENTED_EDGE ( 'NONE', *, *, #27273, .F. ) ;
#65120=FACE_OUTER_BOUND ( 'NONE', #28626, .T. ) ;
#65121=AXIS2_PLACEMENT_3D ( 'NONE', #76361, #58655, #107085 ) ;
#65122=ORIENTED_EDGE ( 'NONE', *, *, #6599, .F. ) ;
#65123=CIRCLE ( 'NONE', #40111, 0.06509327318403745899 ) ;
#65124=CARTESIAN_POINT ( 'NONE',  ( 7.699999999999925571, 2.500000000000000000, 3.883716857408420431 ) ) ;
#65125=EDGE_CURVE ( 'NONE', #17389, #104949, #19350, .T. ) ;
#65126=CARTESIAN_POINT ( 'NONE',  ( 5.449999999999936229, 2.500000000000000000, -2.065063509461102065 ) ) ;
#65127=DIRECTION ( 'NONE',  ( 0.000000000000000000, 0.000000000000000000, -1.000000000000000000 ) ) ;
#65128=ORIENTED_EDGE ( 'NONE', *, *, #38799, .T. ) ;
#65129=CIRCLE ( 'NONE', #23369, 0.06509327318403745899 ) ;
#65130=CARTESIAN_POINT ( 'NONE',  ( -11.84999999999999787, 2.500000000000000000, -1.718653347947321830 ) ) ;
#65131=CARTESIAN_POINT ( 'NONE',  ( 1.449999999999952216, 2.500000000000000000, -2.511473670974877948 ) ) ;
#65132=VERTEX_POINT ( 'NONE', #58059 ) ;
#65133=CARTESIAN_POINT ( 'NONE',  ( -15.79999999999998117, 12.50000000000000000, -0.06509327318403743123 ) ) ;
#65134=ADVANCED_FACE ( 'NONE', ( #127439 ), #128128, .T. ) ;
#65135=ORIENTED_EDGE ( 'NONE', *, *, #106873, .F. ) ;
#65136=VERTEX_POINT ( 'NONE', #118250 ) ;
#65137=DIRECTION ( 'NONE',  ( 0.000000000000000000, 0.000000000000000000, 1.000000000000000000 ) ) ;
#65138=VERTEX_POINT ( 'NONE', #68502 ) ;
#65139=DIRECTION ( 'NONE',  ( 0.000000000000000000, -0.000000000000000000, 1.000000000000000000 ) ) ;
#65140=DIRECTION ( 'NONE',  ( 0.000000000000000000, 0.000000000000000000, -1.000000000000000000 ) ) ;
#65141=LINE ( 'NONE', #27814, #96082 ) ;
#65142=AXIS2_PLACEMENT_3D ( 'NONE', #34577, #25356, #83026 ) ;
#65143=ORIENTED_EDGE ( 'NONE', *, *, #867, .F. ) ;
#65144=AXIS2_PLACEMENT_3D ( 'NONE', #32950, #82686, #24395 ) ;
#65145=FACE_BOUND ( 'NONE', #25145, .T. ) ;
#65146=CARTESIAN_POINT ( 'NONE',  ( -7.300000000000016698, 2.500000000000000000, -4.776537180435978414 ) ) ;
#65147=ORIENTED_EDGE ( 'NONE', *, *, #82727, .T. ) ;
#65148=CARTESIAN_POINT ( 'NONE',  ( 7.699999999999925571, 2.500000000000000000, -4.676537180435978769 ) ) ;
#65149=EDGE_CURVE ( 'NONE', #15822, #16690, #121853, .T. ) ;
#65150=DIRECTION ( 'NONE',  ( 0.000000000000000000, 0.000000000000000000, 1.000000000000000000 ) ) ;
#65151=EDGE_LOOP ( 'NONE', ( #35630, #40820 ) ) ;
#65152=AXIS2_PLACEMENT_3D ( 'NONE', #72989, #25824, #104382 ) ;
#65153=VECTOR ( 'NONE', #99325, 1000.000000000000000 ) ;
#65154=ORIENTED_EDGE ( 'NONE', *, *, #30584, .F. ) ;
#65155=CONICAL_SURFACE ( 'NONE', #8730, 0.1000000000000002554, 0.003490658503988666988 ) ;
#65156=VERTEX_POINT ( 'NONE', #69799 ) ;
#65157=CARTESIAN_POINT ( 'NONE',  ( -3.550000000000028244, 12.50000000000000000, -1.753560074763288679 ) ) ;
#65158=FACE_OUTER_BOUND ( 'NONE', #50418, .T. ) ;
#65159=DIRECTION ( 'NONE',  ( -0.000000000000000000, 1.000000000000000000, -0.000000000000000000 ) ) ;
#65160=FACE_BOUND ( 'NONE', #96811, .T. ) ;
#65161=ORIENTED_EDGE ( 'NONE', *, *, #80300, .F. ) ;
#65163=CARTESIAN_POINT ( 'NONE',  ( -4.600000000000025402, 12.50000000000000000, 4.395220292106234439 ) ) ;
#65164=CARTESIAN_POINT ( 'NONE',  ( -1.450000000000036371, 12.50000000000000000, 6.776507416713035248 ) ) ;
#65165=AXIS2_PLACEMENT_3D ( 'NONE', #118778, #29130, #69023 ) ;
#65166=AXIS2_PLACEMENT_3D ( 'NONE', #25743, #44095, #104311 ) ;
#65168=AXIS2_PLACEMENT_3D ( 'NONE', #76149, #56491, #57146 ) ;
#65169=VECTOR ( 'NONE', #51283, 1000.000000000000000 ) ;
#65170=CIRCLE ( 'NONE', #86099, 0.06509327318403745899 ) ;
#65171=DIRECTION ( 'NONE',  ( 0.000000000000000000, 0.000000000000000000, 1.000000000000000000 ) ) ;
#65172=DIRECTION ( 'NONE',  ( -0.000000000000000000, -1.000000000000000000, -0.000000000000000000 ) ) ;
#65173=DIRECTION ( 'NONE',  ( -0.000000000000000000, -1.000000000000000000, -0.000000000000000000 ) ) ;
#65174=CARTESIAN_POINT ( 'NONE',  ( 0.6499999999999543920, 2.500000000000000000, 6.048780366869521252 ) ) ;
#65175=DIRECTION ( 'NONE',  ( 0.000000000000000000, 0.000000000000000000, 1.000000000000000000 ) ) ;
#65176=EDGE_CURVE ( 'NONE', #30638, #61247, #65419, .T. ) ;
#65177=VERTEX_POINT ( 'NONE', #88114 ) ;
#65178=AXIS2_PLACEMENT_3D ( 'NONE', #120589, #21092, #112063 ) ;
#65179=ORIENTED_EDGE ( 'NONE', *, *, #62771, .T. ) ;
#65180=ORIENTED_EDGE ( 'NONE', *, *, #127946, .T. ) ;
#65181=ORIENTED_EDGE ( 'NONE', *, *, #105170, .F. ) ;
#65182=EDGE_LOOP ( 'NONE', ( #43005, #118966 ) ) ;
#65183=CARTESIAN_POINT ( 'NONE',  ( 0.5999999999999560130, 12.50000000000000000, -3.918623584224389056 ) ) ;
#65184=CARTESIAN_POINT ( 'NONE',  ( 7.949999999999922018, 2.500000000000000000, -2.165063509461101710 ) ) ;
#65185=ORIENTED_EDGE ( 'NONE', *, *, #4742, .F. ) ;
#65186=FACE_BOUND ( 'NONE', #63732, .T. ) ;
#65187=DIRECTION ( 'NONE',  ( 0.000000000000000000, 0.000000000000000000, 1.000000000000000000 ) ) ;
#65188=DIRECTION ( 'NONE',  ( 0.000000000000000000, 0.000000000000000000, 1.000000000000000000 ) ) ;
#65189=VERTEX_POINT ( 'NONE', #108426 ) ;
#65190=ADVANCED_FACE ( 'NONE', ( #109729 ), #59080, .T. ) ;
#65191=CARTESIAN_POINT ( 'NONE',  ( -13.29999999999998828, 12.50000000000000000, 4.330127018922196314 ) ) ;
#65192=ADVANCED_FACE ( 'NONE', ( #107128 ), #15228, .T. ) ;
#65193=DIRECTION ( 'NONE',  ( -0.000000000000000000, -1.000000000000000000, -0.000000000000000000 ) ) ;
#65194=ADVANCED_FACE ( 'NONE', ( #20067 ), #37761, .T. ) ;
#65195=LINE ( 'NONE', #94671, #85136 ) ;
#65196=ADVANCED_FACE ( 'NONE', ( #39726 ), #25608, .T. ) ;
#65197=ORIENTED_EDGE ( 'NONE', *, *, #54598, .F. ) ;
#65198=FACE_OUTER_BOUND ( 'NONE', #43457, .T. ) ;
#65199=ORIENTED_EDGE ( 'NONE', *, *, #29947, .F. ) ;
#65200=EDGE_CURVE ( 'NONE', #128448, #110183, #79998, .T. ) ;
#65201=EDGE_LOOP ( 'NONE', ( #120507, #124427 ) ) ;
#65202=CONICAL_SURFACE ( 'NONE', #2506, 0.1000000000000002554, 0.003490658503988666988 ) ;
#65203=ORIENTED_EDGE ( 'NONE', *, *, #9284, .F. ) ;
#65204=CIRCLE ( 'NONE', #92405, 0.06509327318403745899 ) ;
#65205=CARTESIAN_POINT ( 'NONE',  ( 2.049999999999950084, 12.50000000000000000, -2.165063509461101710 ) ) ;
#65206=CIRCLE ( 'NONE', #54746, 0.06509327318403745899 ) ;
#65207=DIRECTION ( 'NONE',  ( -4.274815082592931898E-19, -0.9999939076577903929, -0.003490651415223739937 ) ) ;
#65209=ORIENTED_EDGE ( 'NONE', *, *, #122767, .F. ) ;
#65210=EDGE_CURVE ( 'NONE', #80531, #125538, #117627, .T. ) ;
#65211=CARTESIAN_POINT ( 'NONE',  ( 13.39473262194674774, 2.500000000000000000, -7.044698189560237189 ) ) ;
#65212=EDGE_CURVE ( 'NONE', #78931, #36319, #17280, .T. ) ;
#65213=DIRECTION ( 'NONE',  ( -0.000000000000000000, -1.000000000000000000, -0.000000000000000000 ) ) ;
#65215=ADVANCED_FACE ( 'NONE', ( #12154 ), #32485, .T. ) ;
#65216=VECTOR ( 'NONE', #26829, 1000.000000000000000 ) ;
#65217=CIRCLE ( 'NONE', #117428, 0.06509327318403745899 ) ;
#65218=FACE_OUTER_BOUND ( 'NONE', #75385, .T. ) ;
#65220=DIRECTION ( 'NONE',  ( 0.000000000000000000, 1.000000000000000000, 0.000000000000000000 ) ) ;
#65221=AXIS2_PLACEMENT_3D ( 'NONE', #114183, #23879, #103727 ) ;
#65222=AXIS2_PLACEMENT_3D ( 'NONE', #85280, #106219, #104904 ) ;
#65223=PLANE ( 'NONE',  #93406 ) ;
#65224=ADVANCED_FACE ( 'NONE', ( #52099 ), #33119, .T. ) ;
#65225=ORIENTED_EDGE ( 'NONE', *, *, #38522, .T. ) ;
#65226=CARTESIAN_POINT ( 'NONE',  ( 5.849999999999933031, 12.50000000000000000, -1.472243186433550122 ) ) ;
#65227=AXIS2_PLACEMENT_3D ( 'NONE', #21496, #11012, #93461 ) ;
#65228=ORIENTED_EDGE ( 'NONE', *, *, #81147, .F. ) ;
#65229=ORIENTED_EDGE ( 'NONE', *, *, #38145, .T. ) ;
#65230=PLANE ( 'NONE',  #24176 ) ;
#65231=DIRECTION ( 'NONE',  ( -0.000000000000000000, -1.000000000000000000, -0.000000000000000000 ) ) ;
#65232=CARTESIAN_POINT ( 'NONE',  ( -9.150000000000009237, 2.500000000000000000, 1.472243186433545459 ) ) ;
#65233=CARTESIAN_POINT ( 'NONE',  ( 12.29999999999990479, 12.50000000000000000, 4.611443907251934426 ) ) ;
#65234=CARTESIAN_POINT ( 'NONE',  ( 4.349999999999936584, 2.500000000000000000, 6.248780366869520542 ) ) ;
#65235=ORIENTED_EDGE ( 'NONE', *, *, #99264, .T. ) ;
#65236=VERTEX_POINT ( 'NONE', #21336 ) ;
#65237=DIRECTION ( 'NONE',  ( 0.000000000000000000, 0.000000000000000000, -1.000000000000000000 ) ) ;
#65238=CARTESIAN_POINT ( 'NONE',  ( 8.099999999999921485, 2.500000000000000000, 0.3464101615137735735 ) ) ;
#65239=FACE_OUTER_BOUND ( 'NONE', #14534, .T. ) ;
#65240=ORIENTED_EDGE ( 'NONE', *, *, #33586, .T. ) ;
#65241=ORIENTED_EDGE ( 'NONE', *, *, #41637, .T. ) ;
#65242=LINE ( 'NONE', #114355, #8088 ) ;
#65243=AXIS2_PLACEMENT_3D ( 'NONE', #16178, #16812, #35845 ) ;
#65244=EDGE_LOOP ( 'NONE', ( #92003, #81114 ) ) ;
#65245=FACE_OUTER_BOUND ( 'NONE', #61304, .T. ) ;
#65246=FACE_OUTER_BOUND ( 'NONE', #30287, .T. ) ;
#65247=VERTEX_POINT ( 'NONE', #61277 ) ;
#65248=LINE ( 'NONE', #67165, #102538 ) ;
#65249=CARTESIAN_POINT ( 'NONE',  ( -5.000000000000022204, 2.500000000000000000, 3.637306695894644726 ) ) ;
#65250=FACE_OUTER_BOUND ( 'NONE', #72966, .T. ) ;
#65251=FACE_OUTER_BOUND ( 'NONE', #88076, .T. ) ;
#65252=AXIS2_PLACEMENT_3D ( 'NONE', #9632, #99951, #10281 ) ;
#65253=ORIENTED_EDGE ( 'NONE', *, *, #61499, .F. ) ;
#65254=AXIS2_PLACEMENT_3D ( 'NONE', #81386, #31629, #71540 ) ;
#65255=ADVANCED_FACE ( 'NONE', ( #60642 ), #98776, .T. ) ;
#65256=VECTOR ( 'NONE', #63038, 1000.000000000000000 ) ;
#65257=FACE_OUTER_BOUND ( 'NONE', #91695, .T. ) ;
#65258=AXIS2_PLACEMENT_3D ( 'NONE', #47290, #54037, #27002 ) ;
#65259=DIRECTION ( 'NONE',  ( 0.000000000000000000, 0.000000000000000000, -1.000000000000000000 ) ) ;
#65260=EDGE_CURVE ( 'NONE', #121148, #24001, #121762, .T. ) ;
#65261=ORIENTED_EDGE ( 'NONE', *, *, #59904, .F. ) ;
#65262=ORIENTED_EDGE ( 'NONE', *, *, #11742, .T. ) ;
#65263=CARTESIAN_POINT ( 'NONE',  ( -5.600000000000020073, 12.50000000000000000, 0.3464101615137736845 ) ) ;
#65264=PLANE ( 'NONE',  #103448 ) ;
#65265=FACE_OUTER_BOUND ( 'NONE', #10870, .T. ) ;
#65266=DIRECTION ( 'NONE',  ( -0.000000000000000000, 1.000000000000000000, -0.000000000000000000 ) ) ;
#65267=CONICAL_SURFACE ( 'NONE', #82005, 0.1000000000000002554, 0.003490658503988666988 ) ;
#65268=LINE ( 'NONE', #95392, #113801 ) ;
#65269=EDGE_CURVE ( 'NONE', #54407, #14513, #105127, .T. ) ;
#65270=DIRECTION ( 'NONE',  ( 0.000000000000000000, 0.000000000000000000, 1.000000000000000000 ) ) ;
#65271=CIRCLE ( 'NONE', #52754, 0.06509327318403745899 ) ;
#65272=DIRECTION ( 'NONE',  ( -4.274815082592931898E-19, -0.9999939076577903929, -0.003490651415223739937 ) ) ;
#65274=DIRECTION ( 'NONE',  ( -0.000000000000000000, -1.000000000000000000, -0.000000000000000000 ) ) ;
#65275=CIRCLE ( 'NONE', #25556, 0.06509327318403745899 ) ;
#65276=CARTESIAN_POINT ( 'NONE',  ( 8.149999999999923972, 2.500000000000000000, 1.718653347947321386 ) ) ;
#65277=CIRCLE ( 'NONE', #10880, 0.1000000000000000056 ) ;
#65278=CARTESIAN_POINT ( 'NONE',  ( 4.599999999999938360, 2.500000000000000000, -0.6928203230275541413 ) ) ;
#65279=AXIS2_PLACEMENT_3D ( 'NONE', #57636, #68732, #98832 ) ;
#65280=CARTESIAN_POINT ( 'NONE',  ( 12.09999999999990550, 2.500000000000000000, 5.122947341949749323 ) ) ;
#65281=VERTEX_POINT ( 'NONE', #112309 ) ;
#65282=AXIS2_PLACEMENT_3D ( 'NONE', #56191, #35916, #43831 ) ;
#65283=ORIENTED_EDGE ( 'NONE', *, *, #39284, .T. ) ;
#65284=ORIENTED_EDGE ( 'NONE', *, *, #36588, .F. ) ;
#65285=DIRECTION ( 'NONE',  ( 0.000000000000000000, 0.000000000000000000, 1.000000000000000000 ) ) ;
#65286=DIRECTION ( 'NONE',  ( 0.000000000000000000, 1.000000000000000000, 0.000000000000000000 ) ) ;
#65287=DIRECTION ( 'NONE',  ( 0.000000000000000000, 1.000000000000000000, 0.000000000000000000 ) ) ;
#65288=ORIENTED_EDGE ( 'NONE', *, *, #51657, .T. ) ;
#65289=CARTESIAN_POINT ( 'NONE',  ( 18.09027855933934603, -2.526462839860887488, -2.685672775344543961 ) ) ;
#65290=CARTESIAN_POINT ( 'NONE',  ( 11.44999999999990870, 12.50000000000000000, 6.906693963081109722 ) ) ;
#65291=DIRECTION ( 'NONE',  ( 0.000000000000000000, 0.000000000000000000, -1.000000000000000000 ) ) ;
#65292=ORIENTED_EDGE ( 'NONE', *, *, #109740, .F. ) ;
#65293=DIRECTION ( 'NONE',  ( -0.000000000000000000, -1.000000000000000000, -0.000000000000000000 ) ) ;
#65294=EDGE_LOOP ( 'NONE', ( #56545, #55188, #126323, #54785 ) ) ;
#65295=ORIENTED_EDGE ( 'NONE', *, *, #19444, .T. ) ;
#65297=CIRCLE ( 'NONE', #73709, 0.06509327318403745899 ) ;
#65298=ORIENTED_EDGE ( 'NONE', *, *, #87831, .F. ) ;
#65299=CARTESIAN_POINT ( 'NONE',  ( 5.449999999999936229, 2.500000000000000000, -2.265063509461101798 ) ) ;
#65300=AXIS2_PLACEMENT_3D ( 'NONE', #4512, #53012, #3264 ) ;
#65301=CIRCLE ( 'NONE', #40289, 0.09999999999999999167 ) ;
#65302=DIRECTION ( 'NONE',  ( 0.000000000000000000, 0.000000000000000000, 1.000000000000000000 ) ) ;
#65303=CARTESIAN_POINT ( 'NONE',  ( 5.599999999999933031, 12.50000000000000000, -0.3464101615137783474 ) ) ;
#65304=CARTESIAN_POINT ( 'NONE',  ( 3.549999999999944755, 12.50000000000000000, -6.841600689897077814 ) ) ;
#65305=CONICAL_SURFACE ( 'NONE', #38136, 0.1000000000000002554, 0.003490658503988666988 ) ;
#65306=VERTEX_POINT ( 'NONE', #92016 ) ;
#65307=CIRCLE ( 'NONE', #111270, 0.09999999999999982514 ) ;
#65308=AXIS2_PLACEMENT_3D ( 'NONE', #91654, #82497, #81824 ) ;
#65309=DIRECTION ( 'NONE',  ( 0.000000000000000000, 0.000000000000000000, 1.000000000000000000 ) ) ;
#65310=CIRCLE ( 'NONE', #46531, 0.1000000000000000056 ) ;
#65311=EDGE_CURVE ( 'NONE', #27245, #125732, #75787, .T. ) ;
#65312=ORIENTED_EDGE ( 'NONE', *, *, #99833, .T. ) ;
#65313=CARTESIAN_POINT ( 'NONE',  ( 87.50000000000001421, -3.974992050023849810, -6.359987280038161828 ) ) ;
#65314=DIRECTION ( 'NONE',  ( -0.000000000000000000, -1.000000000000000000, -0.000000000000000000 ) ) ;
#65315=VECTOR ( 'NONE', #24850, 1000.000000000000000 ) ;
#65316=CARTESIAN_POINT ( 'NONE',  ( 8.349999999999919709, 12.50000000000000000, 6.560283801567334372 ) ) ;
#65317=CARTESIAN_POINT ( 'NONE',  ( 17.29982614914667849, -2.489966891809442195, 2.989943721779569241 ) ) ;
#65318=EDGE_CURVE ( 'NONE', #24755, #115443, #41656, .T. ) ;
#65319=AXIS2_PLACEMENT_3D ( 'NONE', #70447, #11520, #2998 ) ;
#65320=ORIENTED_EDGE ( 'NONE', *, *, #15271, .T. ) ;
#65321=ORIENTED_EDGE ( 'NONE', *, *, #13755, .T. ) ;
#65322=ORIENTED_EDGE ( 'NONE', *, *, #72214, .T. ) ;
#65323=CARTESIAN_POINT ( 'NONE',  ( -5.000000000000022204, 2.500000000000000000, 3.737306695894644371 ) ) ;
#65324=PLANE ( 'NONE',  #39445 ) ;
#65325=EDGE_CURVE ( 'NONE', #93435, #65003, #13083, .T. ) ;
#65326=CARTESIAN_POINT ( 'NONE',  ( 10.19999999999991225, 12.50000000000000000, 3.983716857408420076 ) ) ;
#65327=FACE_BOUND ( 'NONE', #64112, .T. ) ;
#65328=LINE ( 'NONE', #85623, #26406 ) ;
#65329=DIRECTION ( 'NONE',  ( 0.000000000000000000, 1.000000000000000000, 0.000000000000000000 ) ) ;
#65330=DIRECTION ( 'NONE',  ( -0.000000000000000000, -1.000000000000000000, -0.000000000000000000 ) ) ;
#65331=CARTESIAN_POINT ( 'NONE',  ( -13.14999999999999147, 2.500000000000000000, -1.918653347947324006 ) ) ;
#65332=AXIS2_PLACEMENT_3D ( 'NONE', #55978, #76277, #67066 ) ;
#65334=CARTESIAN_POINT ( 'NONE',  ( 14.79999999999989235, 12.50000000000000000, 0.4115034346978109769 ) ) ;
#65335=LINE ( 'NONE', #66630, #78451 ) ;
#65336=AXIS2_PLACEMENT_3D ( 'NONE', #106358, #115512, #27788 ) ;
#65337=CIRCLE ( 'NONE', #96730, 0.06509327318403745899 ) ;
#65338=VECTOR ( 'NONE', #2742, 1000.000000000000000 ) ;
#65339=DIRECTION ( 'NONE',  ( 0.000000000000000000, 0.000000000000000000, 1.000000000000000000 ) ) ;
#65340=EDGE_CURVE ( 'NONE', #46062, #29998, #100539, .T. ) ;
#65342=ORIENTED_EDGE ( 'NONE', *, *, #122220, .F. ) ;
#65343=ORIENTED_EDGE ( 'NONE', *, *, #52322, .F. ) ;
#65345=DIRECTION ( 'NONE',  ( 0.000000000000000000, 1.000000000000000000, 0.000000000000000000 ) ) ;
#65346=FACE_BOUND ( 'NONE', #82000, .T. ) ;
#65347=CIRCLE ( 'NONE', #52743, 0.06509327318403745899 ) ;
#65348=CARTESIAN_POINT ( 'NONE',  ( -13.29999999999999005, 12.50000000000000000, 1.843143693225357538E-15 ) ) ;
#65349=AXIS2_PLACEMENT_3D ( 'NONE', #53797, #24985, #112733 ) ;
#65350=EDGE_CURVE ( 'NONE', #7100, #60983, #109234, .T. ) ;
#65351=ORIENTED_EDGE ( 'NONE', *, *, #55916, .T. ) ;
#65352=EDGE_CURVE ( 'NONE', #60457, #26852, #86243, .T. ) ;
#65353=CARTESIAN_POINT ( 'NONE',  ( 43.31961220463728068, 2.029667686321675824, 5.113275312219439428 ) ) ;
#65354=EDGE_CURVE ( 'NONE', #42353, #40264, #40355, .T. ) ;
#65355=CARTESIAN_POINT ( 'NONE',  ( -9.999999999999969802, 12.50000000000000000, 4.330127018922196314 ) ) ;
#65356=EDGE_CURVE ( 'NONE', #120673, #9996, #12789, .T. ) ;
#65357=ADVANCED_FACE ( 'NONE', ( #1054 ), #107181, .T. ) ;
#65358=ORIENTED_EDGE ( 'NONE', *, *, #110647, .T. ) ;
#65359=CARTESIAN_POINT ( 'NONE',  ( 5.849999999999934808, 2.500000000000000000, -5.702370205355749455 ) ) ;
#65360=DIRECTION ( 'NONE',  ( -4.274815082592931898E-19, -0.9999939076577903929, -0.003490651415223739937 ) ) ;
#65361=AXIS2_PLACEMENT_3D ( 'NONE', #75980, #28833, #119774 ) ;
#65362=AXIS2_PLACEMENT_3D ( 'NONE', #18890, #128886, #107922 ) ;
#65363=AXIS2_PLACEMENT_3D ( 'NONE', #117089, #27424, #7793 ) ;
#65364=CIRCLE ( 'NONE', #92567, 0.06509327318403745899 ) ;
#65365=ADVANCED_FACE ( 'NONE', ( #80271 ), #67448, .T. ) ;
#65366=ORIENTED_EDGE ( 'NONE', *, *, #21182, .T. ) ;
#65367=FACE_OUTER_BOUND ( 'NONE', #48200, .T. ) ;
#65368=EDGE_CURVE ( 'NONE', #111104, #17511, #123911, .T. ) ;
#65369=LINE ( 'NONE', #105310, #1545 ) ;
#65370=VECTOR ( 'NONE', #123622, 1000.000000000000000 ) ;
#65371=ADVANCED_FACE ( 'NONE', ( #110988 ), #23660, .T. ) ;
#65372=EDGE_LOOP ( 'NONE', ( #4731, #61921, #125451, #38658 ) ) ;
#65373=DIRECTION ( 'NONE',  ( -0.000000000000000000, 1.000000000000000000, -0.000000000000000000 ) ) ;
#65374=EDGE_CURVE ( 'NONE', #91777, #41716, #98866, .T. ) ;
#65375=CIRCLE ( 'NONE', #92579, 0.06509327318403745899 ) ;
#65376=CARTESIAN_POINT ( 'NONE',  ( 11.64999999999990798, 12.50000000000000000, 7.122917578226811486 ) ) ;
#65377=CARTESIAN_POINT ( 'NONE',  ( -10.85000000000000142, 2.500000000000000000, -2.165063509461097713 ) ) ;
#65378=ORIENTED_EDGE ( 'NONE', *, *, #10791, .F. ) ;
#65379=VERTEX_POINT ( 'NONE', #76724 ) ;
#65380=CARTESIAN_POINT ( 'NONE',  ( 5.649999999999936406, 2.500000000000000000, -6.148780366869526226 ) ) ;
#65381=EDGE_CURVE ( 'NONE', #78182, #126113, #34134, .T. ) ;
#65382=VERTEX_POINT ( 'NONE', #125185 ) ;
#65384=CARTESIAN_POINT ( 'NONE',  ( 13.94999999999989448, 2.500000000000000000, -2.511473670974877948 ) ) ;
#65385=DIRECTION ( 'NONE',  ( 0.000000000000000000, 1.000000000000000000, 0.000000000000000000 ) ) ;
#65386=EDGE_LOOP ( 'NONE', ( #78873, #9570, #92639, #105057 ) ) ;
#65387=LINE ( 'NONE', #6438, #58055 ) ;
#65388=CARTESIAN_POINT ( 'NONE',  ( -9.200000000000009948, 2.500000000000000000, -4.330127018922197202 ) ) ;
#65389=CARTESIAN_POINT ( 'NONE',  ( -4.550000000000026468, 12.50000000000000000, -6.495190528383302464 ) ) ;
#65390=AXIS2_PLACEMENT_3D ( 'NONE', #63498, #112604, #62850 ) ;
#65391=CARTESIAN_POINT ( 'NONE',  ( 8.749999999999920064, 2.500000000000000000, -2.857883832488653741 ) ) ;
#65392=AXIS2_PLACEMENT_3D ( 'NONE', #108605, #28774, #7818 ) ;
#65393=CARTESIAN_POINT ( 'NONE',  ( 6.249999999999930722, 12.50000000000000000, -1.472243186433550122 ) ) ;
#65394=ORIENTED_EDGE ( 'NONE', *, *, #37784, .F. ) ;
#65395=EDGE_LOOP ( 'NONE', ( #31144, #32101 ) ) ;
#65396=CARTESIAN_POINT ( 'NONE',  ( 7.899999999999924860, 2.500000000000000000, -4.330127018922201643 ) ) ;
#65397=AXIS2_PLACEMENT_3D ( 'NONE', #26684, #96689, #56758 ) ;
#65398=CARTESIAN_POINT ( 'NONE',  ( 19.09982477502536113, -0.5559300837585569033, 4.454172625795894014 ) ) ;
#65399=CIRCLE ( 'NONE', #109319, 0.1000000000000002554 ) ;
#65400=VECTOR ( 'NONE', #68987, 1000.000000000000000 ) ;
#65401=DIRECTION ( 'NONE',  ( -0.000000000000000000, 1.000000000000000000, -0.000000000000000000 ) ) ;
#65402=ORIENTED_EDGE ( 'NONE', *, *, #110090, .F. ) ;
#65403=ORIENTED_EDGE ( 'NONE', *, *, #102791, .T. ) ;
#65404=VERTEX_POINT ( 'NONE', #56428 ) ;
#65405=DIRECTION ( 'NONE',  ( 0.000000000000000000, 0.000000000000000000, 1.000000000000000000 ) ) ;
#65406=DIRECTION ( 'NONE',  ( -0.000000000000000000, -1.000000000000000000, -0.000000000000000000 ) ) ;
#65407=CIRCLE ( 'NONE', #98852, 0.09999999999999982514 ) ;
#65408=CONICAL_SURFACE ( 'NONE', #84288, 0.1000000000000002554, 0.003490658503988666988 ) ;
#65410=CIRCLE ( 'NONE', #36190, 0.06509327318403745899 ) ;
#65411=CARTESIAN_POINT ( 'NONE',  ( 2.899999999999945732, 2.500000000000000000, -4.330127018922201643 ) ) ;
#65412=CARTESIAN_POINT ( 'NONE',  ( -6.250000000000017764, 2.500000000000000000, 2.857883832488649301 ) ) ;
#65414=CIRCLE ( 'NONE', #121758, 0.1000000000000002554 ) ;
#65415=DIRECTION ( 'NONE',  ( -0.000000000000000000, -1.000000000000000000, -0.000000000000000000 ) ) ;
#65416=FACE_OUTER_BOUND ( 'NONE', #125707, .T. ) ;
#65417=AXIS2_PLACEMENT_3D ( 'NONE', #63333, #101333, #111114 ) ;
#65418=DIRECTION ( 'NONE',  ( -4.274815082592931898E-19, -0.9999939076577903929, -0.003490651415223739937 ) ) ;
#65419=CIRCLE ( 'NONE', #8886, 0.06509327318403745899 ) ;
#65420=ORIENTED_EDGE ( 'NONE', *, *, #62783, .F. ) ;
#65421=EDGE_CURVE ( 'NONE', #65795, #117086, #4864, .T. ) ;
#65422=ADVANCED_FACE ( 'NONE', ( #68178 ), #6906, .T. ) ;
#65423=CARTESIAN_POINT ( 'NONE',  ( -0.8000000000000376810, 2.500000000000000000, -4.230127018922201998 ) ) ;
#65424=VERTEX_POINT ( 'NONE', #116640 ) ;
#65425=ORIENTED_EDGE ( 'NONE', *, *, #37059, .T. ) ;
#65426=DIRECTION ( 'NONE',  ( 0.000000000000000000, 0.000000000000000000, 1.000000000000000000 ) ) ;
#65427=CARTESIAN_POINT ( 'NONE',  ( 8.099999999999923261, 12.50000000000000000, -4.676537180435978769 ) ) ;
#65428=DIRECTION ( 'NONE',  ( 0.000000000000000000, 0.000000000000000000, 1.000000000000000000 ) ) ;
#65429=AXIS2_PLACEMENT_3D ( 'NONE', #10580, #39452, #50518 ) ;
#65430=DIRECTION ( 'NONE',  ( -0.000000000000000000, 1.000000000000000000, -0.000000000000000000 ) ) ;
#65431=CARTESIAN_POINT ( 'NONE',  ( -10.65000000000000213, 12.50000000000000000, 1.883746621131358934 ) ) ;
#65432=DIRECTION ( 'NONE',  ( 0.000000000000000000, -0.000000000000000000, 1.000000000000000000 ) ) ;
#65433=DIRECTION ( 'NONE',  ( 0.000000000000000000, 0.000000000000000000, 1.000000000000000000 ) ) ;
#65434=ORIENTED_EDGE ( 'NONE', *, *, #78900, .F. ) ;
#65435=CARTESIAN_POINT ( 'NONE',  ( -1.650000000000034772, 2.500000000000000000, 5.802370205355744659 ) ) ;
#65436=CIRCLE ( 'NONE', #40328, 0.1000000000000002554 ) ;
#65437=CARTESIAN_POINT ( 'NONE',  ( -7.100000000000017408, 2.500000000000000000, 0.6928203230275494784 ) ) ;
#65438=VERTEX_POINT ( 'NONE', #108110 ) ;
#65439=CONICAL_SURFACE ( 'NONE', #54977, 0.09999999999999982514, 0.003490658503988666988 ) ;
#65440=ORIENTED_EDGE ( 'NONE', *, *, #101270, .T. ) ;
#65441=ORIENTED_EDGE ( 'NONE', *, *, #55319, .F. ) ;
#65442=VERTEX_POINT ( 'NONE', #86538 ) ;
#65443=CONICAL_SURFACE ( 'NONE', #61263, 0.09999999999999999167, 0.003490658503988666988 ) ;
#65444=DIRECTION ( 'NONE',  ( 0.000000000000000000, 1.000000000000000000, 0.000000000000000000 ) ) ;
#65445=DIRECTION ( 'NONE',  ( -0.000000000000000000, -1.000000000000000000, -0.000000000000000000 ) ) ;
#65446=AXIS2_PLACEMENT_3D ( 'NONE', #45649, #124198, #126780 ) ;
#65447=AXIS2_PLACEMENT_3D ( 'NONE', #29500, #20324, #81176 ) ;
#65448=LINE ( 'NONE', #105385, #86136 ) ;
#65449=CARTESIAN_POINT ( 'NONE',  ( -3.350000000000028955, 12.50000000000000000, -2.165063509461101710 ) ) ;
#65450=CARTESIAN_POINT ( 'NONE',  ( 10.39999999999991331, 12.50000000000000000, -2.385244779468109755E-15 ) ) ;
#65451=EDGE_LOOP ( 'NONE', ( #70241, #23678, #66662, #69218 ) ) ;
#65452=CARTESIAN_POINT ( 'NONE',  ( 2.899999999999946620, 12.50000000000000000, -5.088040615133791356 ) ) ;
#65453=CARTESIAN_POINT ( 'NONE',  ( -3.749999999999991118, 2.500000000000000000, 2.165063509461097713 ) ) ;
#65454=CIRCLE ( 'NONE', #42208, 0.1000000000000002554 ) ;
#65455=DIRECTION ( 'NONE',  ( -0.000000000000000000, 1.000000000000000000, -0.000000000000000000 ) ) ;
#65456=EDGE_CURVE ( 'NONE', #117955, #30611, #6652, .T. ) ;
#65457=VERTEX_POINT ( 'NONE', #36811 ) ;
#65458=CIRCLE ( 'NONE', #94809, 0.06509327318403745899 ) ;
#65459=CIRCLE ( 'NONE', #55107, 0.1000000000000002554 ) ;
#65460=AXIS2_PLACEMENT_3D ( 'NONE', #122889, #11635, #50931 ) ;
#65461=ORIENTED_EDGE ( 'NONE', *, *, #44535, .F. ) ;
#65462=EDGE_LOOP ( 'NONE', ( #65515, #68371 ) ) ;
#65463=CARTESIAN_POINT ( 'NONE',  ( -3.750000000000027978, 2.500000000000000000, 7.288010851410849256 ) ) ;
#65464=CIRCLE ( 'NONE', #52963, 0.06509327318403745899 ) ;
#65465=CARTESIAN_POINT ( 'NONE',  ( 0.4499999999999569344, 2.500000000000000000, -2.165063509461101710 ) ) ;
#65466=FACE_OUTER_BOUND ( 'NONE', #74177, .T. ) ;
#65467=CIRCLE ( 'NONE', #121625, 0.06509327318403745899 ) ;
#65468=EDGE_CURVE ( 'NONE', #125450, #120640, #46650, .T. ) ;
#65469=ORIENTED_EDGE ( 'NONE', *, *, #82750, .F. ) ;
#65470=DIRECTION ( 'NONE',  ( 0.000000000000000000, 0.000000000000000000, 1.000000000000000000 ) ) ;
#65471=CARTESIAN_POINT ( 'NONE',  ( -9.600000000000006750, 2.500000000000000000, 4.922947341949748257 ) ) ;
#65472=DIRECTION ( 'NONE',  ( 0.000000000000000000, 1.000000000000000000, 0.000000000000000000 ) ) ;
#65473=DIRECTION ( 'NONE',  ( -0.000000000000000000, 1.000000000000000000, -0.000000000000000000 ) ) ;
#65474=EDGE_CURVE ( 'NONE', #60587, #102800, #50855, .T. ) ;
#65475=CARTESIAN_POINT ( 'NONE',  ( -3.550000000000031797, 12.50000000000000000, -6.148780366869526226 ) ) ;
#65476=ORIENTED_EDGE ( 'NONE', *, *, #71560, .F. ) ;
#65477=DIRECTION ( 'NONE',  ( 0.000000000000000000, 0.000000000000000000, 1.000000000000000000 ) ) ;
#65478=EDGE_LOOP ( 'NONE', ( #65378, #284, #50462, #61048 ) ) ;
#65479=VERTEX_POINT ( 'NONE', #75422 ) ;
#65480=CONICAL_SURFACE ( 'NONE', #4837, 0.09999999999999982514, 0.003490658503988666988 ) ;
#65482=AXIS2_PLACEMENT_3D ( 'NONE', #40622, #32729, #92928 ) ;
#65484=DIRECTION ( 'NONE',  ( 0.000000000000000000, 0.000000000000000000, -1.000000000000000000 ) ) ;
#65485=FACE_BOUND ( 'NONE', #8722, .T. ) ;
#65486=CARTESIAN_POINT ( 'NONE',  ( 4.599999999999939249, 2.500000000000000000, -3.737306695894649700 ) ) ;
#65487=FACE_OUTER_BOUND ( 'NONE', #109839, .T. ) ;
#65488=DIRECTION ( 'NONE',  ( -4.274815082592931898E-19, -0.9999939076577903929, -0.003490651415223739937 ) ) ;
#65489=AXIS2_PLACEMENT_3D ( 'NONE', #37838, #108510, #116390 ) ;
#65490=AXIS2_PLACEMENT_3D ( 'NONE', #82697, #102326, #92490 ) ;
#65491=ORIENTED_EDGE ( 'NONE', *, *, #3758, .T. ) ;
#65492=DIRECTION ( 'NONE',  ( 0.000000000000000000, 1.000000000000000000, 0.000000000000000000 ) ) ;
#65493=CARTESIAN_POINT ( 'NONE',  ( 13.74999999999993072, 2.500000000000000000, -2.265063509461101798 ) ) ;
#65494=DIRECTION ( 'NONE',  ( -0.000000000000000000, -1.000000000000000000, -0.000000000000000000 ) ) ;
#65495=CARTESIAN_POINT ( 'NONE',  ( 7.099999999999926814, 12.50000000000000000, -0.6928203230275541413 ) ) ;
#65496=ORIENTED_EDGE ( 'NONE', *, *, #73953, .T. ) ;
#65497=AXIS2_PLACEMENT_3D ( 'NONE', #73350, #92343, #23616 ) ;
#65499=AXIS2_PLACEMENT_3D ( 'NONE', #120631, #88593, #40141 ) ;
#65500=AXIS2_PLACEMENT_3D ( 'NONE', #122034, #121372, #12065 ) ;
#65501=FACE_OUTER_BOUND ( 'NONE', #95545, .T. ) ;
#65502=VECTOR ( 'NONE', #42398, 1000.000000000000000 ) ;
#65503=VERTEX_POINT ( 'NONE', #57069 ) ;
#65504=CONICAL_SURFACE ( 'NONE', #44588, 0.1000000000000002554, 0.003490658503988666988 ) ;
#65505=DIRECTION ( 'NONE',  ( -4.274815082592931898E-19, -0.9999939076577903929, -0.003490651415223739937 ) ) ;
#65506=ORIENTED_EDGE ( 'NONE', *, *, #39437, .F. ) ;
#65507=FACE_BOUND ( 'NONE', #70545, .T. ) ;
#65508=AXIS2_PLACEMENT_3D ( 'NONE', #39406, #41331, #111310 ) ;
#65509=DIRECTION ( 'NONE',  ( 0.000000000000000000, 0.000000000000000000, -1.000000000000000000 ) ) ;
#65510=ADVANCED_FACE ( 'NONE', ( #97648 ), #42462, .T. ) ;
#65511=VERTEX_POINT ( 'NONE', #27600 ) ;
#65512=CARTESIAN_POINT ( 'NONE',  ( 9.599999999999914380, 12.50000000000000000, 3.637306695894644726 ) ) ;
#65513=DIRECTION ( 'NONE',  ( 0.000000000000000000, 0.000000000000000000, 1.000000000000000000 ) ) ;
#65514=EDGE_LOOP ( 'NONE', ( #12394, #115274 ) ) ;
#65515=ORIENTED_EDGE ( 'NONE', *, *, #116206, .F. ) ;
#65516=EDGE_CURVE ( 'NONE', #49071, #104330, #97005, .T. ) ;
#65518=EDGE_CURVE ( 'NONE', #55213, #23957, #57107, .T. ) ;
#65519=ORIENTED_EDGE ( 'NONE', *, *, #20204, .F. ) ;
#65521=LINE ( 'NONE', #15769, #21932 ) ;
#65522=FACE_OUTER_BOUND ( 'NONE', #36960, .T. ) ;
#65523=DIRECTION ( 'NONE',  ( -4.274815082592931898E-19, -0.9999939076577903929, -0.003490651415223739937 ) ) ;
#65524=ADVANCED_FACE ( 'NONE', ( #95728 ), #127129, .T. ) ;
#65526=DIRECTION ( 'NONE',  ( 0.000000000000000000, 1.000000000000000000, 0.000000000000000000 ) ) ;
#65527=ADVANCED_FACE ( 'NONE', ( #76083 ), #73834, .T. ) ;
#65528=AXIS2_PLACEMENT_3D ( 'NONE', #112061, #82609, #70201 ) ;
#65529=AXIS2_PLACEMENT_3D ( 'NONE', #106384, #44904, #65150 ) ;
#65530=ORIENTED_EDGE ( 'NONE', *, *, #57183, .F. ) ;
#65532=FACE_OUTER_BOUND ( 'NONE', #123982, .T. ) ;
#65533=EDGE_CURVE ( 'NONE', #43052, #74901, #115582, .T. ) ;
#65534=DIRECTION ( 'NONE',  ( -4.274815082592931898E-19, -0.9999939076577903929, -0.003490651415223739937 ) ) ;
#65535=CARTESIAN_POINT ( 'NONE',  ( -7.900000000000011013, 2.500000000000000000, 4.330127018922196314 ) ) ;
#65536=DIRECTION ( 'NONE',  ( -0.000000000000000000, 1.000000000000000000, -0.000000000000000000 ) ) ;
#65537=ORIENTED_EDGE ( 'NONE', *, *, #117578, .T. ) ;
#65538=VERTEX_POINT ( 'NONE', #118569 ) ;
#65539=FACE_BOUND ( 'NONE', #30419, .T. ) ;
#65540=ORIENTED_EDGE ( 'NONE', *, *, #9480, .F. ) ;
#65541=CIRCLE ( 'NONE', #67584, 0.06509327318403745899 ) ;
#65542=DIRECTION ( 'NONE',  ( -0.000000000000000000, -1.000000000000000000, -0.000000000000000000 ) ) ;
#65543=DIRECTION ( 'NONE',  ( 0.000000000000000000, -0.9999939076577903929, 0.003490651415223739937 ) ) ;
#65544=AXIS2_PLACEMENT_3D ( 'NONE', #51455, #100525, #2312 ) ;
#65545=EDGE_CURVE ( 'NONE', #72858, #102123, #28928, .T. ) ;
#65546=ORIENTED_EDGE ( 'NONE', *, *, #58044, .F. ) ;
#65547=PLANE ( 'NONE',  #24210 ) ;
#65548=DIRECTION ( 'NONE',  ( -4.274815082592931898E-19, -0.9999939076577903929, -0.003490651415223739937 ) ) ;
#65549=AXIS2_PLACEMENT_3D ( 'NONE', #68528, #58084, #106045 ) ;
#65550=LINE ( 'NONE', #123813, #22136 ) ;
#65551=DIRECTION ( 'NONE',  ( 0.000000000000000000, 0.000000000000000000, -1.000000000000000000 ) ) ;
#65552=DIRECTION ( 'NONE',  ( -0.000000000000000000, 1.000000000000000000, -0.000000000000000000 ) ) ;
#65553=CARTESIAN_POINT ( 'NONE',  ( -9.550000000000002487, 2.500000000000000000, 6.495190528383297135 ) ) ;
#65555=FACE_OUTER_BOUND ( 'NONE', #63706, .T. ) ;
#65556=DIRECTION ( 'NONE',  ( 0.000000000000000000, 1.000000000000000000, 0.000000000000000000 ) ) ;
#65557=EDGE_LOOP ( 'NONE', ( #55635, #80282 ) ) ;
#65558=ORIENTED_EDGE ( 'NONE', *, *, #43878, .F. ) ;
#65559=CARTESIAN_POINT ( 'NONE',  ( -12.49999999999999289, 2.500000000000000000, 3.537306695894645081 ) ) ;
#65560=AXIS2_PLACEMENT_3D ( 'NONE', #963, #40923, #80829 ) ;
#65561=EDGE_LOOP ( 'NONE', ( #86771, #28666, #33601, #92035 ) ) ;
#65562=CONICAL_SURFACE ( 'NONE', #113687, 0.1000000000000002554, 0.003490658503988666988 ) ;
#65563=DIRECTION ( 'NONE',  ( 0.000000000000000000, -0.9999939076577903929, 0.003490651415223739937 ) ) ;
#65564=VERTEX_POINT ( 'NONE', #120518 ) ;
#65565=VERTEX_POINT ( 'NONE', #728 ) ;
#65566=EDGE_LOOP ( 'NONE', ( #42195, #105537 ) ) ;
#65567=AXIS2_PLACEMENT_3D ( 'NONE', #28516, #118819, #108348 ) ;
#65568=CARTESIAN_POINT ( 'NONE',  ( 12.09999999999990550, 12.50000000000000000, 5.022947341949748790 ) ) ;
#65569=CONICAL_SURFACE ( 'NONE', #88544, 0.09999999999999982514, 0.003490658503988666988 ) ;
#65570=PLANE ( 'NONE',  #853 ) ;
#65571=CARTESIAN_POINT ( 'NONE',  ( 5.599999999999931255, 2.500000000000000000, 4.676537180435972552 ) ) ;
#65572=DIRECTION ( 'NONE',  ( 0.000000000000000000, 0.000000000000000000, 1.000000000000000000 ) ) ;
#65573=PLANE ( 'NONE',  #12031 ) ;
#65574=ORIENTED_EDGE ( 'NONE', *, *, #102644, .T. ) ;
#65575=DIRECTION ( 'NONE',  ( -0.000000000000000000, -1.000000000000000000, -0.000000000000000000 ) ) ;
#65576=ORIENTED_EDGE ( 'NONE', *, *, #101620, .F. ) ;
#65577=VERTEX_POINT ( 'NONE', #48559 ) ;
#65578=ORIENTED_EDGE ( 'NONE', *, *, #87524, .T. ) ;
#65579=EDGE_CURVE ( 'NONE', #93847, #87716, #75889, .T. ) ;
#65580=VERTEX_POINT ( 'NONE', #81241 ) ;
#65581=DIRECTION ( 'NONE',  ( 0.000000000000000000, 0.000000000000000000, -1.000000000000000000 ) ) ;
#65582=AXIS2_PLACEMENT_3D ( 'NONE', #51602, #33870, #31959 ) ;
#65583=CIRCLE ( 'NONE', #9150, 0.1000000000000002554 ) ;
#65584=ORIENTED_EDGE ( 'NONE', *, *, #66726, .F. ) ;
#65585=ORIENTED_EDGE ( 'NONE', *, *, #73783, .T. ) ;
#65587=ADVANCED_FACE ( 'NONE', ( #30864 ), #109398, .T. ) ;
#65588=CARTESIAN_POINT ( 'NONE',  ( 0.6499999999999561684, 2.500000000000000000, 1.918653347947321564 ) ) ;
#65589=CIRCLE ( 'NONE', #111559, 0.06509327318403745899 ) ;
#65590=FACE_OUTER_BOUND ( 'NONE', #20786, .T. ) ;
#65591=CIRCLE ( 'NONE', #124177, 0.1000000000000000472 ) ;
#65592=DIRECTION ( 'NONE',  ( 0.000000000000000000, 0.000000000000000000, 1.000000000000000000 ) ) ;
#65593=CARTESIAN_POINT ( 'NONE',  ( -4.800000000000028244, 12.50000000000000000, -4.048810130592463530 ) ) ;
#65594=AXIS2_PLACEMENT_3D ( 'NONE', #109399, #97006, #98285 ) ;
#65595=CARTESIAN_POINT ( 'NONE',  ( -1.450000000000035927, 2.500000000000000000, -1.918653347947326004 ) ) ;
#65596=ORIENTED_EDGE ( 'NONE', *, *, #39230, .T. ) ;
#65597=DIRECTION ( 'NONE',  ( 0.000000000000000000, 0.000000000000000000, -1.000000000000000000 ) ) ;
#65598=VECTOR ( 'NONE', #3189, 1000.000000000000000 ) ;
#65599=CIRCLE ( 'NONE', #25893, 0.1000000000000000472 ) ;
#65600=ORIENTED_EDGE ( 'NONE', *, *, #113424, .F. ) ;
#65601=DIRECTION ( 'NONE',  ( -4.274815082592931898E-19, -0.9999939076577903929, -0.003490651415223739937 ) ) ;
#65602=EDGE_LOOP ( 'NONE', ( #92384, #29594 ) ) ;
#65603=PLANE ( 'NONE',  #104643 ) ;
#65604=ORIENTED_EDGE ( 'NONE', *, *, #15385, .T. ) ;
#65605=AXIS2_PLACEMENT_3D ( 'NONE', #79300, #40016, #60928 ) ;
#65606=ORIENTED_EDGE ( 'NONE', *, *, #50425, .T. ) ;
#65607=CARTESIAN_POINT ( 'NONE',  ( -0.8500000000000386136, 2.500000000000000000, 2.757883832488649656 ) ) ;
#65608=DIRECTION ( 'NONE',  ( 0.000000000000000000, 0.000000000000000000, -1.000000000000000000 ) ) ;
#65609=DIRECTION ( 'NONE',  ( 0.000000000000000000, 0.000000000000000000, 1.000000000000000000 ) ) ;
#65610=CARTESIAN_POINT ( 'NONE',  ( -13.14999999999999147, 2.500000000000000000, 2.511473670974877503 ) ) ;
#65611=CARTESIAN_POINT ( 'NONE',  ( -13.29999999999999005, 2.500000000000000000, -4.430127018922199511 ) ) ;
#65612=ORIENTED_EDGE ( 'NONE', *, *, #28602, .T. ) ;
#65613=CARTESIAN_POINT ( 'NONE',  ( -1.250000000000035749, 2.500000000000000000, -2.957883832488653830 ) ) ;
#65614=CARTESIAN_POINT ( 'NONE',  ( 6.049999999999934097, 2.500000000000000000, -2.511473670974877948 ) ) ;
#65615=FACE_OUTER_BOUND ( 'NONE', #41756, .T. ) ;
#65616=DIRECTION ( 'NONE',  ( 0.000000000000000000, 0.000000000000000000, -1.000000000000000000 ) ) ;
#65617=AXIS2_PLACEMENT_3D ( 'NONE', #129117, #108788, #8645 ) ;
#65618=CARTESIAN_POINT ( 'NONE',  ( -10.40000000000000213, 2.500000000000000000, 4.330127018922196314 ) ) ;
#65619=ADVANCED_FACE ( 'NONE', ( #59019 ), #666, .T. ) ;
#65620=EDGE_LOOP ( 'NONE', ( #35308, #67285 ) ) ;
#65621=EDGE_LOOP ( 'NONE', ( #67465, #84148 ) ) ;
#65622=ORIENTED_EDGE ( 'NONE', *, *, #64965, .T. ) ;
#65623=AXIS2_PLACEMENT_3D ( 'NONE', #13188, #95001, #115915 ) ;
#65624=DIRECTION ( 'NONE',  ( -0.000000000000000000, 1.000000000000000000, -0.000000000000000000 ) ) ;
#65625=DIRECTION ( 'NONE',  ( 0.000000000000000000, 0.000000000000000000, -1.000000000000000000 ) ) ;
#65626=EDGE_CURVE ( 'NONE', #32850, #56986, #82159, .T. ) ;
#65627=CIRCLE ( 'NONE', #99094, 0.06509327318403743123 ) ;
#65628=EDGE_CURVE ( 'NONE', #35861, #121566, #119223, .T. ) ;
#65630=PLANE ( 'NONE',  #92892 ) ;
#65631=CARTESIAN_POINT ( 'NONE',  ( -9.200000000000006395, 12.50000000000000000, -0.06509327318403980434 ) ) ;
#65632=DIRECTION ( 'NONE',  ( 0.000000000000000000, 1.000000000000000000, 0.000000000000000000 ) ) ;
#65633=EDGE_CURVE ( 'NONE', #73190, #60441, #21677, .T. ) ;
#65635=ORIENTED_EDGE ( 'NONE', *, *, #46632, .T. ) ;
#65636=AXIS2_PLACEMENT_3D ( 'NONE', #15966, #44154, #83454 ) ;
#65637=VECTOR ( 'NONE', #20730, 1000.000000000000000 ) ;
#65638=DIRECTION ( 'NONE',  ( 0.000000000000000000, 0.000000000000000000, -1.000000000000000000 ) ) ;
#65639=CARTESIAN_POINT ( 'NONE',  ( 8.099999999999923261, 2.500000000000000000, 4.776537180435972196 ) ) ;
#65640=EDGE_CURVE ( 'NONE', #7221, #36118, #92619, .T. ) ;
#65641=ORIENTED_EDGE ( 'NONE', *, *, #110875, .F. ) ;
#65642=EDGE_CURVE ( 'NONE', #74504, #59695, #27867, .T. ) ;
#65643=DIRECTION ( 'NONE',  ( 0.000000000000000000, 1.000000000000000000, 0.000000000000000000 ) ) ;
#65644=DIRECTION ( 'NONE',  ( 0.000000000000000000, 0.000000000000000000, -1.000000000000000000 ) ) ;
#65645=DIRECTION ( 'NONE',  ( 0.000000000000000000, 0.000000000000000000, 1.000000000000000000 ) ) ;
#65646=ORIENTED_EDGE ( 'NONE', *, *, #76209, .F. ) ;
#65647=VECTOR ( 'NONE', #28323, 1000.000000000000000 ) ;
#65648=AXIS2_PLACEMENT_3D ( 'NONE', #33994, #32724, #73911 ) ;
#65649=LINE ( 'NONE', #28313, #59450 ) ;
#65651=AXIS2_PLACEMENT_3D ( 'NONE', #75505, #105631, #74879 ) ;
#65652=ORIENTED_EDGE ( 'NONE', *, *, #85886, .T. ) ;
#65653=LINE ( 'NONE', #96388, #73053 ) ;
#65654=DIRECTION ( 'NONE',  ( 0.000000000000000000, -0.9999939076577903929, 0.003490651415223739937 ) ) ;
#65655=VERTEX_POINT ( 'NONE', #70768 ) ;
#65656=DIRECTION ( 'NONE',  ( 0.000000000000000000, 1.000000000000000000, 0.000000000000000000 ) ) ;
#65657=CARTESIAN_POINT ( 'NONE',  ( -2.950000000000030376, 2.500000000000000000, 6.495190528383297135 ) ) ;
#65658=ORIENTED_EDGE ( 'NONE', *, *, #108769, .F. ) ;
#65659=CARTESIAN_POINT ( 'NONE',  ( -5.850000000000018296, 2.500000000000000000, 7.088010851410848190 ) ) ;
#65660=ORIENTED_EDGE ( 'NONE', *, *, #15713, .T. ) ;
#65661=ORIENTED_EDGE ( 'NONE', *, *, #95416, .F. ) ;
#65662=CARTESIAN_POINT ( 'NONE',  ( 3.749999999999940492, 2.500000000000000000, 2.957883832488649389 ) ) ;
#65663=CARTESIAN_POINT ( 'NONE',  ( 11.84999999999990372, 2.500000000000000000, 1.918653347947321564 ) ) ;
#65664=AXIS2_PLACEMENT_3D ( 'NONE', #35829, #14861, #94737 ) ;
#65665=AXIS2_PLACEMENT_3D ( 'NONE', #99895, #10220, #90052 ) ;
#65666=VERTEX_POINT ( 'NONE', #110684 ) ;
#65667=DIRECTION ( 'NONE',  ( 0.000000000000000000, 1.000000000000000000, 0.000000000000000000 ) ) ;
#65668=DIRECTION ( 'NONE',  ( 0.000000000000000000, 0.000000000000000000, -1.000000000000000000 ) ) ;
#65669=ORIENTED_EDGE ( 'NONE', *, *, #16984, .F. ) ;
#65670=EDGE_CURVE ( 'NONE', #126920, #56076, #78041, .T. ) ;
#65671=CARTESIAN_POINT ( 'NONE',  ( 8.149999999999923972, 2.500000000000000000, 1.818653347947321475 ) ) ;
#65672=DIRECTION ( 'NONE',  ( 0.000000000000000000, 0.000000000000000000, -1.000000000000000000 ) ) ;
#65673=CIRCLE ( 'NONE', #88668, 0.09999999999999982514 ) ;
#65674=VECTOR ( 'NONE', #111067, 1000.000000000000000 ) ;
#65675=CIRCLE ( 'NONE', #99054, 0.06509327318403745899 ) ;
#65676=EDGE_CURVE ( 'NONE', #24152, #79929, #21606, .T. ) ;
#65677=DIRECTION ( 'NONE',  ( 0.000000000000000000, -0.000000000000000000, 1.000000000000000000 ) ) ;
#65678=LINE ( 'NONE', #125878, #78057 ) ;
#65679=ADVANCED_FACE ( 'NONE', ( #40030 ), #48812, .T. ) ;
#65680=CARTESIAN_POINT ( 'NONE',  ( 13.14999999999989733, 2.500000000000000000, -2.411473670974877859 ) ) ;
#65681=DIRECTION ( 'NONE',  ( 0.000000000000000000, 0.000000000000000000, -1.000000000000000000 ) ) ;
#65682=EDGE_CURVE ( 'NONE', #77485, #59628, #9082, .T. ) ;
#65683=EDGE_CURVE ( 'NONE', #63939, #7340, #8977, .T. ) ;
#65684=CIRCLE ( 'NONE', #11401, 0.06509327318403745899 ) ;
#65685=AXIS2_PLACEMENT_3D ( 'NONE', #40094, #57804, #80011 ) ;
#65686=VERTEX_POINT ( 'NONE', #88460 ) ;
#65687=VERTEX_POINT ( 'NONE', #128429 ) ;
#65688=EDGE_CURVE ( 'NONE', #91704, #41081, #38763, .T. ) ;
#65689=ORIENTED_EDGE ( 'NONE', *, *, #25472, .T. ) ;
#65690=VERTEX_POINT ( 'NONE', #4570 ) ;
#65691=CARTESIAN_POINT ( 'NONE',  ( 4.599999999999936584, 12.50000000000000000, 4.265033745738159077 ) ) ;
#65692=CARTESIAN_POINT ( 'NONE',  ( -7.100000000000017408, 2.500000000000000000, 0.6928203230275494784 ) ) ;
#65693=CIRCLE ( 'NONE', #120086, 0.1000000000000002554 ) ;
#65694=CARTESIAN_POINT ( 'NONE',  ( 9.999999999999911182, 2.500000000000000000, -3.637306695894650055 ) ) ;
#65695=EDGE_LOOP ( 'NONE', ( #73721, #1416 ) ) ;
#65696=FACE_BOUND ( 'NONE', #113856, .T. ) ;
#65697=LINE ( 'NONE', #85966, #96009 ) ;
#65698=FACE_OUTER_BOUND ( 'NONE', #110980, .T. ) ;
#65699=EDGE_CURVE ( 'NONE', #12208, #21956, #102789, .T. ) ;
#65700=DIRECTION ( 'NONE',  ( -0.000000000000000000, 1.000000000000000000, -0.000000000000000000 ) ) ;
#65702=FACE_OUTER_BOUND ( 'NONE', #58367, .T. ) ;
#65703=CARTESIAN_POINT ( 'NONE',  ( 0.6499999999999566125, 2.500000000000000000, -6.048780366869526581 ) ) ;
#65704=CARTESIAN_POINT ( 'NONE',  ( -0.4500000000000402012, 2.500000000000000000, 6.495190528383297135 ) ) ;
#65705=FACE_OUTER_BOUND ( 'NONE', #118834, .T. ) ;
#65706=DIRECTION ( 'NONE',  ( 0.000000000000000000, 0.000000000000000000, 1.000000000000000000 ) ) ;
#65707=CARTESIAN_POINT ( 'NONE',  ( 6.449999999999930012, 2.500000000000000000, 6.841600689897072485 ) ) ;
#65708=CIRCLE ( 'NONE', #117935, 0.1000000000000000472 ) ;
#65709=CARTESIAN_POINT ( 'NONE',  ( -7.900000000000014566, 12.50000000000000000, -3.702399969078687292 ) ) ;
#65710=EDGE_LOOP ( 'NONE', ( #1328, #61412 ) ) ;
#65711=VERTEX_POINT ( 'NONE', #34076 ) ;
#65713=EDGE_LOOP ( 'NONE', ( #89784, #117437, #60032, #98612 ) ) ;
#65714=CARTESIAN_POINT ( 'NONE',  ( -9.150000000000009237, 12.50000000000000000, -2.165063509461101710 ) ) ;
#65715=VERTEX_POINT ( 'NONE', #124389 ) ;
#65716=FACE_OUTER_BOUND ( 'NONE', #18734, .T. ) ;
#65717=ORIENTED_EDGE ( 'NONE', *, *, #71860, .T. ) ;
#65718=EDGE_CURVE ( 'NONE', #107053, #63043, #456, .T. ) ;
#65719=ORIENTED_EDGE ( 'NONE', *, *, #7723, .T. ) ;
#65720=CARTESIAN_POINT ( 'NONE',  ( -5.850000000000021849, 2.500000000000000000, -2.857883832488653741 ) ) ;
#65721=VECTOR ( 'NONE', #51680, 1000.000000000000000 ) ;
#65722=FACE_OUTER_BOUND ( 'NONE', #100672, .T. ) ;
#65723=CARTESIAN_POINT ( 'NONE',  ( -10.00000000000000533, 2.500000000000000000, 5.122947341949749323 ) ) ;
#65724=DIRECTION ( 'NONE',  ( 0.000000000000000000, 0.000000000000000000, -1.000000000000000000 ) ) ;
#65725=FACE_OUTER_BOUND ( 'NONE', #88962, .T. ) ;
#65726=ORIENTED_EDGE ( 'NONE', *, *, #17925, .T. ) ;
#65727=ORIENTED_EDGE ( 'NONE', *, *, #52677, .T. ) ;
#65728=CIRCLE ( 'NONE', #67785, 0.06509327318403745899 ) ;
#65729=ORIENTED_EDGE ( 'NONE', *, *, #118604, .F. ) ;
#65730=EDGE_LOOP ( 'NONE', ( #75130, #53837 ) ) ;
#65731=DIRECTION ( 'NONE',  ( -0.000000000000000000, 1.000000000000000000, -0.000000000000000000 ) ) ;
#65732=EDGE_LOOP ( 'NONE', ( #29905, #19041 ) ) ;
#65733=ORIENTED_EDGE ( 'NONE', *, *, #50090, .F. ) ;
#65734=DIRECTION ( 'NONE',  ( 0.000000000000000000, 0.000000000000000000, 1.000000000000000000 ) ) ;
#65735=EDGE_CURVE ( 'NONE', #108831, #53510, #50658, .T. ) ;
#65737=CIRCLE ( 'NONE', #74060, 0.06509327318403745899 ) ;
#65738=DIRECTION ( 'NONE',  ( 0.000000000000000000, -0.000000000000000000, 1.000000000000000000 ) ) ;
#65739=VECTOR ( 'NONE', #76971, 1000.000000000000000 ) ;
#65740=DIRECTION ( 'NONE',  ( -0.000000000000000000, 1.000000000000000000, -0.000000000000000000 ) ) ;
#65741=DIRECTION ( 'NONE',  ( 0.000000000000000000, -0.9999939076577903929, 0.003490651415223739937 ) ) ;
#65743=ORIENTED_EDGE ( 'NONE', *, *, #86142, .T. ) ;
#65744=AXIS2_PLACEMENT_3D ( 'NONE', #75016, #26560, #95940 ) ;
#65745=FACE_OUTER_BOUND ( 'NONE', #68572, .T. ) ;
#65746=ORIENTED_EDGE ( 'NONE', *, *, #91933, .F. ) ;
#65747=DIRECTION ( 'NONE',  ( 0.000000000000000000, 0.000000000000000000, 1.000000000000000000 ) ) ;
#65748=ORIENTED_EDGE ( 'NONE', *, *, #49141, .F. ) ;
#65749=DIRECTION ( 'NONE',  ( 0.000000000000000000, -0.000000000000000000, 1.000000000000000000 ) ) ;
#65750=CARTESIAN_POINT ( 'NONE',  ( 11.64999999999990798, 12.50000000000000000, -2.857883832488653741 ) ) ;
#65751=ORIENTED_EDGE ( 'NONE', *, *, #34227, .T. ) ;
#65752=DIRECTION ( 'NONE',  ( -0.000000000000000000, -1.000000000000000000, -0.000000000000000000 ) ) ;
#65753=CARTESIAN_POINT ( 'NONE',  ( -1.850000000000033396, 2.500000000000000000, -1.818653347947325916 ) ) ;
#65754=ORIENTED_EDGE ( 'NONE', *, *, #80592, .F. ) ;
#65755=DIRECTION ( 'NONE',  ( 0.000000000000000000, 0.000000000000000000, 1.000000000000000000 ) ) ;
#65756=AXIS2_PLACEMENT_3D ( 'NONE', #89437, #48224, #129395 ) ;
#65757=DIRECTION ( 'NONE',  ( 0.000000000000000000, 1.000000000000000000, 0.000000000000000000 ) ) ;
#65758=EDGE_LOOP ( 'NONE', ( #81921, #69246, #44149, #12260 ) ) ;
#65759=CONICAL_SURFACE ( 'NONE', #17727, 0.1000000000000002554, 0.003490658503988666988 ) ;
#65760=CIRCLE ( 'NONE', #51207, 0.09999999999999982514 ) ;
#65761=ORIENTED_EDGE ( 'NONE', *, *, #67403, .F. ) ;
#65762=DIRECTION ( 'NONE',  ( 0.000000000000000000, -0.9999939076577903929, 0.003490651415223739937 ) ) ;
#65763=CARTESIAN_POINT ( 'NONE',  ( -3.950000000000024603, 2.500000000000000000, -2.611473670974877592 ) ) ;
#65766=CIRCLE ( 'NONE', #9339, 0.06509327318403745899 ) ;
#65767=CARTESIAN_POINT ( 'NONE',  ( 12.09999999999990550, 12.50000000000000000, -5.088040615133791356 ) ) ;
#65768=CIRCLE ( 'NONE', #95308, 0.06509327318403743123 ) ;
#65769=CIRCLE ( 'NONE', #76155, 0.09999999999999982514 ) ;
#65770=DIRECTION ( 'NONE',  ( 0.000000000000000000, 0.000000000000000000, 1.000000000000000000 ) ) ;
#65771=VECTOR ( 'NONE', #69982, 1000.000000000000000 ) ;
#65772=EDGE_CURVE ( 'NONE', #65023, #14140, #73628, .T. ) ;
#65773=EDGE_LOOP ( 'NONE', ( #104865, #92647 ) ) ;
#65774=VECTOR ( 'NONE', #84920, 1000.000000000000000 ) ;
#65775=CARTESIAN_POINT ( 'NONE',  ( 76.44832593087598127, 3.583109180387994641, -6.086770968619237721 ) ) ;
#65776=AXIS2_PLACEMENT_3D ( 'NONE', #110604, #2561, #32068 ) ;
#65777=ADVANCED_FACE ( 'NONE', ( #111991 ), #6705, .T. ) ;
#65778=ORIENTED_EDGE ( 'NONE', *, *, #68618, .F. ) ;
#65780=EDGE_CURVE ( 'NONE', #115619, #48060, #115682, .T. ) ;
#65781=DIRECTION ( 'NONE',  ( 0.000000000000000000, -0.9999939076577903929, 0.003490651415223739937 ) ) ;
#65783=CARTESIAN_POINT ( 'NONE',  ( 5.599999999999931255, 2.500000000000000000, 4.576537180435972019 ) ) ;
#65784=EDGE_CURVE ( 'NONE', #31107, #57789, #111184, .T. ) ;
#65785=ORIENTED_EDGE ( 'NONE', *, *, #28178, .F. ) ;
#65786=DIRECTION ( 'NONE',  ( -0.000000000000000000, 1.000000000000000000, -0.000000000000000000 ) ) ;
#65787=CARTESIAN_POINT ( 'NONE',  ( 6.249999999999967137, 2.500000000000000000, 6.395190528383296602 ) ) ;
#65788=EDGE_CURVE ( 'NONE', #59434, #74772, #98665, .T. ) ;
#65789=EDGE_CURVE ( 'NONE', #103313, #62839, #74631, .T. ) ;
#65790=EDGE_CURVE ( 'NONE', #75929, #126716, #109124, .T. ) ;
#65791=EDGE_CURVE ( 'NONE', #20224, #116295, #92710, .T. ) ;
#65792=VERTEX_POINT ( 'NONE', #24248 ) ;
#65793=CARTESIAN_POINT ( 'NONE',  ( 5.849999999999933920, 2.500000000000000000, 5.802370205355744659 ) ) ;
#65794=ORIENTED_EDGE ( 'NONE', *, *, #99411, .T. ) ;
#65795=VERTEX_POINT ( 'NONE', #53066 ) ;
#65796=CARTESIAN_POINT ( 'NONE',  ( -4.600000000000024514, 2.500000000000000000, 0.6928203230275494784 ) ) ;
#65797=EDGE_CURVE ( 'NONE', #39483, #36299, #92997, .T. ) ;
#65798=ORIENTED_EDGE ( 'NONE', *, *, #118861, .T. ) ;
#65799=DIRECTION ( 'NONE',  ( 0.000000000000000000, -0.9999939076577903929, 0.003490651415223739937 ) ) ;
#65800=CARTESIAN_POINT ( 'NONE',  ( -8.350000000000008527, 2.500000000000000000, 7.288010851410849256 ) ) ;
#65801=CIRCLE ( 'NONE', #86737, 0.1000000000000002554 ) ;
#65802=CARTESIAN_POINT ( 'NONE',  ( -7.500000000000001776, 2.500000000000000000, 1.734723475976807094E-15 ) ) ;
#65804=ORIENTED_EDGE ( 'NONE', *, *, #128347, .T. ) ;
#65805=FACE_BOUND ( 'NONE', #90017, .T. ) ;
#65806=DIRECTION ( 'NONE',  ( -0.000000000000000000, -1.000000000000000000, -0.000000000000000000 ) ) ;
#65807=VERTEX_POINT ( 'NONE', #103457 ) ;
#65809=CARTESIAN_POINT ( 'NONE',  ( 1.649999999999951061, 2.500000000000000000, -6.595190528383302109 ) ) ;
#65810=EDGE_LOOP ( 'NONE', ( #10655, #52644, #112805, #34401 ) ) ;
#65811=AXIS2_PLACEMENT_3D ( 'NONE', #87851, #38126, #117962 ) ;
#65812=ORIENTED_EDGE ( 'NONE', *, *, #106401, .T. ) ;
#65813=CONICAL_SURFACE ( 'NONE', #9407, 0.1000000000000002554, 0.003490658503988666988 ) ;
#65814=EDGE_LOOP ( 'NONE', ( #93252, #37701, #43753, #67512 ) ) ;
#65815=CARTESIAN_POINT ( 'NONE',  ( -8.550000000000014921, 2.500000000000000000, -6.148780366869520897 ) ) ;
#65816=CARTESIAN_POINT ( 'NONE',  ( 4.849235612604186230, 2.499999999999999112, 8.943930330504295867 ) ) ;
#65817=DIRECTION ( 'NONE',  ( 0.000000000000000000, 0.000000000000000000, 1.000000000000000000 ) ) ;
#65818=EDGE_CURVE ( 'NONE', #117733, #102950, #38050, .T. ) ;
#65819=FACE_BOUND ( 'NONE', #30590, .T. ) ;
#65820=ORIENTED_EDGE ( 'NONE', *, *, #17935, .T. ) ;
#65822=CARTESIAN_POINT ( 'NONE',  ( 6.849999999999929479, 2.500000000000000000, -1.818653347947326138 ) ) ;
#65823=DIRECTION ( 'NONE',  ( 0.000000000000000000, -0.9999939076577903929, 0.003490651415223739937 ) ) ;
#65824=DIRECTION ( 'NONE',  ( 0.000000000000000000, 1.000000000000000000, 0.000000000000000000 ) ) ;
#65825=CONICAL_SURFACE ( 'NONE', #21945, 0.09999999999999982514, 0.003490658503988666988 ) ;
#65826=VECTOR ( 'NONE', #122693, 1000.000000000000000 ) ;
#65827=LINE ( 'NONE', #6248, #69504 ) ;
#65828=CARTESIAN_POINT ( 'NONE',  ( -7.700000000000010836, 2.500000000000000000, 4.083716857408421497 ) ) ;
#65830=DIRECTION ( 'NONE',  ( 0.000000000000000000, -0.000000000000000000, 1.000000000000000000 ) ) ;
#65831=DIRECTION ( 'NONE',  ( -0.000000000000000000, -1.000000000000000000, -0.000000000000000000 ) ) ;
#65832=EDGE_CURVE ( 'NONE', #109827, #84019, #2827, .T. ) ;
#65833=DIRECTION ( 'NONE',  ( 0.000000000000000000, 1.000000000000000000, 0.000000000000000000 ) ) ;
#65834=EDGE_CURVE ( 'NONE', #1184, #12403, #75681, .T. ) ;
#65835=ORIENTED_EDGE ( 'NONE', *, *, #47010, .F. ) ;
#65836=ORIENTED_EDGE ( 'NONE', *, *, #68744, .T. ) ;
#65837=ORIENTED_EDGE ( 'NONE', *, *, #38903, .F. ) ;
#65838=ORIENTED_EDGE ( 'NONE', *, *, #45035, .T. ) ;
#65839=ORIENTED_EDGE ( 'NONE', *, *, #35063, .F. ) ;
#65840=LINE ( 'NONE', #36411, #4569 ) ;
#65841=LINE ( 'NONE', #16722, #88542 ) ;
#65842=EDGE_LOOP ( 'NONE', ( #99702, #80801, #82707, #86091 ) ) ;
#65843=EDGE_CURVE ( 'NONE', #121535, #60091, #107076, .T. ) ;
#65844=FACE_BOUND ( 'NONE', #117063, .T. ) ;
#65845=AXIS2_PLACEMENT_3D ( 'NONE', #60910, #92299, #2620 ) ;
#65846=DIRECTION ( 'NONE',  ( -0.000000000000000000, 1.000000000000000000, -0.000000000000000000 ) ) ;
#65847=EDGE_CURVE ( 'NONE', #4275, #42483, #2651, .T. ) ;
#65848=EDGE_CURVE ( 'NONE', #63445, #74853, #67346, .T. ) ;
#65849=EDGE_CURVE ( 'NONE', #51178, #90407, #42259, .T. ) ;
#65850=CONICAL_SURFACE ( 'NONE', #120244, 0.1000000000000002554, 0.003490658503988666988 ) ;
#65851=DIRECTION ( 'NONE',  ( 0.000000000000000000, 1.000000000000000000, 0.000000000000000000 ) ) ;
#65852=VECTOR ( 'NONE', #7491, 1000.000000000000000 ) ;
#65853=CIRCLE ( 'NONE', #103519, 0.06509327318403745899 ) ;
#65854=DIRECTION ( 'NONE',  ( 0.000000000000000000, 0.000000000000000000, 1.000000000000000000 ) ) ;
#65855=DIRECTION ( 'NONE',  ( 0.000000000000000000, 0.000000000000000000, -1.000000000000000000 ) ) ;
#65856=CARTESIAN_POINT ( 'NONE',  ( 5.399999999999932854, 12.50000000000000000, 3.637306695894644726 ) ) ;
#65857=ORIENTED_EDGE ( 'NONE', *, *, #119176, .F. ) ;
#65858=CARTESIAN_POINT ( 'NONE',  ( -0.6000000000000323963, 2.500000000000000000, -0.3464101615137759604 ) ) ;
#65859=EDGE_CURVE ( 'NONE', #69451, #114181, #15028, .T. ) ;
#65860=VECTOR ( 'NONE', #121945, 1000.000000000000000 ) ;
#65861=ORIENTED_EDGE ( 'NONE', *, *, #72836, .F. ) ;
#65862=CIRCLE ( 'NONE', #36554, 0.06509327318403745899 ) ;
#65863=CONICAL_SURFACE ( 'NONE', #90912, 0.1000000000000002554, 0.003490658503988666988 ) ;
#65865=EDGE_LOOP ( 'NONE', ( #100056, #54942 ) ) ;
#65866=CARTESIAN_POINT ( 'NONE',  ( -5.000000000000026645, 12.50000000000000000, -3.637306695894650055 ) ) ;
#65867=VECTOR ( 'NONE', #126162, 1000.000000000000000 ) ;
#65868=FACE_OUTER_BOUND ( 'NONE', #105657, .T. ) ;
#65869=DIRECTION ( 'NONE',  ( 0.000000000000000000, 0.000000000000000000, -1.000000000000000000 ) ) ;
#65870=VERTEX_POINT ( 'NONE', #57589 ) ;
#65871=CARTESIAN_POINT ( 'NONE',  ( 14.38463633656722607, 2.500000000000127454, -7.683002074691031247 ) ) ;
#65872=AXIS2_PLACEMENT_3D ( 'NONE', #85412, #124703, #24561 ) ;
#65873=VECTOR ( 'NONE', #14648, 1000.000000000000000 ) ;
#65874=PLANE ( 'NONE',  #82513 ) ;
#65875=DIRECTION ( 'NONE',  ( 0.000000000000000000, 0.000000000000000000, 1.000000000000000000 ) ) ;
#65877=CARTESIAN_POINT ( 'NONE',  ( -10.65000000000000391, 2.500000000000000000, -1.818653347947322141 ) ) ;
#65878=VECTOR ( 'NONE', #123877, 1000.000000000000000 ) ;
#65879=CARTESIAN_POINT ( 'NONE',  ( -12.49999999999999289, 2.500000000000000000, 3.737306695894644371 ) ) ;
#65881=DIRECTION ( 'NONE',  ( 0.000000000000000000, 1.000000000000000000, 0.000000000000000000 ) ) ;
#65882=ORIENTED_EDGE ( 'NONE', *, *, #89004, .T. ) ;
#65883=VERTEX_POINT ( 'NONE', #106031 ) ;
#65885=FACE_OUTER_BOUND ( 'NONE', #9978, .T. ) ;
#65886=CARTESIAN_POINT ( 'NONE',  ( 5.849999999999933920, 2.500000000000000000, -2.957883832488653830 ) ) ;
#65887=CIRCLE ( 'NONE', #74216, 0.1000000000000002554 ) ;
#65888=EDGE_LOOP ( 'NONE', ( #35509, #110766 ) ) ;
#65889=ORIENTED_EDGE ( 'NONE', *, *, #97382, .F. ) ;
#65891=ADVANCED_FACE ( 'NONE', ( #45830 ), #125649, .T. ) ;
#65892=DIRECTION ( 'NONE',  ( 0.000000000000000000, 0.000000000000000000, -1.000000000000000000 ) ) ;
#65893=DIRECTION ( 'NONE',  ( 0.000000000000000000, 1.000000000000000000, 0.000000000000000000 ) ) ;
#65894=EDGE_LOOP ( 'NONE', ( #5387, #114053 ) ) ;
#65895=ORIENTED_EDGE ( 'NONE', *, *, #109737, .T. ) ;
#65896=DIRECTION ( 'NONE',  ( 0.000000000000000000, 0.000000000000000000, 1.000000000000000000 ) ) ;
#65897=CONICAL_SURFACE ( 'NONE', #49207, 0.1000000000000002554, 0.003490658503988666988 ) ;
#65898=CIRCLE ( 'NONE', #61727, 0.1000000000000000472 ) ;
#65899=ORIENTED_EDGE ( 'NONE', *, *, #62821, .T. ) ;
#65900=DIRECTION ( 'NONE',  ( -0.000000000000000000, -1.000000000000000000, -0.000000000000000000 ) ) ;
#65901=VECTOR ( 'NONE', #123459, 1000.000000000000000 ) ;
#65902=DIRECTION ( 'NONE',  ( 0.000000000000000000, 0.000000000000000000, 1.000000000000000000 ) ) ;
#65903=VERTEX_POINT ( 'NONE', #96841 ) ;
#65904=FACE_OUTER_BOUND ( 'NONE', #95739, .T. ) ;
#65905=DIRECTION ( 'NONE',  ( -0.000000000000000000, 1.000000000000000000, -0.000000000000000000 ) ) ;
#65906=FACE_OUTER_BOUND ( 'NONE', #23046, .T. ) ;
#65907=ADVANCED_FACE ( 'NONE', ( #27449 ), #56892, .T. ) ;
#65908=FACE_OUTER_BOUND ( 'NONE', #72306, .T. ) ;
#65909=EDGE_LOOP ( 'NONE', ( #28652, #117612 ) ) ;
#65910=AXIS2_PLACEMENT_3D ( 'NONE', #63571, #34110, #51823 ) ;
#65911=CARTESIAN_POINT ( 'NONE',  ( -8.950000000000009948, 2.500000000000000000, -6.841600689897072485 ) ) ;
#65912=DIRECTION ( 'NONE',  ( 0.000000000000000000, 1.000000000000000000, 0.000000000000000000 ) ) ;
#65913=AXIS2_PLACEMENT_3D ( 'NONE', #2407, #10935, #90814 ) ;
#65914=ORIENTED_EDGE ( 'NONE', *, *, #3891, .F. ) ;
#65915=ORIENTED_EDGE ( 'NONE', *, *, #32128, .F. ) ;
#65917=DIRECTION ( 'NONE',  ( 0.000000000000000000, 0.000000000000000000, -1.000000000000000000 ) ) ;
#65918=LINE ( 'NONE', #25341, #105428 ) ;
#65919=DIRECTION ( 'NONE',  ( 0.000000000000000000, 0.000000000000000000, 1.000000000000000000 ) ) ;
#65920=DIRECTION ( 'NONE',  ( 0.000000000000000000, 0.000000000000000000, -1.000000000000000000 ) ) ;
#65921=CARTESIAN_POINT ( 'NONE',  ( -2.050000000000032685, 12.50000000000000000, -6.560283801567339701 ) ) ;
#65922=AXIS2_PLACEMENT_3D ( 'NONE', #41555, #81468, #82101 ) ;
#65923=AXIS2_PLACEMENT_3D ( 'NONE', #34336, #93883, #66341 ) ;
#65924=CARTESIAN_POINT ( 'NONE',  ( -8.350000000000012079, 2.500000000000000000, 2.857883832488649301 ) ) ;
#65925=FACE_OUTER_BOUND ( 'NONE', #82570, .T. ) ;
#65926=CARTESIAN_POINT ( 'NONE',  ( -11.24999999999999822, 2.500000000000000000, 1.472243186433545459 ) ) ;
#65928=EDGE_LOOP ( 'NONE', ( #58768, #75160, #9540, #6092 ) ) ;
#65929=EDGE_CURVE ( 'NONE', #60457, #38221, #47763, .T. ) ;
#65930=VECTOR ( 'NONE', #61389, 1000.000000000000000 ) ;
#65931=EDGE_LOOP ( 'NONE', ( #80713, #100716 ) ) ;
#65932=DIRECTION ( 'NONE',  ( -0.000000000000000000, -1.000000000000000000, -0.000000000000000000 ) ) ;
#65933=ORIENTED_EDGE ( 'NONE', *, *, #109566, .T. ) ;
#65934=FACE_OUTER_BOUND ( 'NONE', #99161, .T. ) ;
#65935=AXIS2_PLACEMENT_3D ( 'NONE', #49027, #8422, #48361 ) ;
#65936=DIRECTION ( 'NONE',  ( -0.000000000000000000, -1.000000000000000000, -0.000000000000000000 ) ) ;
#65937=DIRECTION ( 'NONE',  ( -4.274815082592931898E-19, -0.9999939076577903929, -0.003490651415223739937 ) ) ;
#65938=ADVANCED_FACE ( 'NONE', ( #35365 ), #27647, .T. ) ;
#65940=DIRECTION ( 'NONE',  ( -0.000000000000000000, -1.000000000000000000, -0.000000000000000000 ) ) ;
#65941=AXIS2_PLACEMENT_3D ( 'NONE', #54189, #64002, #42441 ) ;
#65942=CIRCLE ( 'NONE', #63895, 0.09999999999999982514 ) ;
#65943=CARTESIAN_POINT ( 'NONE',  ( 8.349999999999919709, 2.500000000000000000, -2.165063509461101710 ) ) ;
#65944=DIRECTION ( 'NONE',  ( 0.000000000000000000, 1.000000000000000000, 0.000000000000000000 ) ) ;
#65945=ORIENTED_EDGE ( 'NONE', *, *, #67483, .T. ) ;
#65946=EDGE_CURVE ( 'NONE', #82878, #22551, #58982, .T. ) ;
#65947=EDGE_CURVE ( 'NONE', #110204, #90702, #47123, .T. ) ;
#65948=EDGE_CURVE ( 'NONE', #38247, #37082, #63178, .T. ) ;
#65949=EDGE_CURVE ( 'NONE', #104107, #107896, #52710, .T. ) ;
#65950=EDGE_CURVE ( 'NONE', #76636, #116200, #19245, .T. ) ;
#65951=DIRECTION ( 'NONE',  ( -0.000000000000000000, 1.000000000000000000, -0.000000000000000000 ) ) ;
#65952=ORIENTED_EDGE ( 'NONE', *, *, #115920, .F. ) ;
#65953=AXIS2_PLACEMENT_3D ( 'NONE', #123859, #123240, #33573 ) ;
#65954=EDGE_LOOP ( 'NONE', ( #104353, #75305, #2694, #8702 ) ) ;
#65956=ORIENTED_EDGE ( 'NONE', *, *, #84326, .F. ) ;
#65957=DIRECTION ( 'NONE',  ( 0.000000000000000000, 1.000000000000000000, 0.000000000000000000 ) ) ;
#65958=VECTOR ( 'NONE', #52123, 1000.000000000000000 ) ;
#65959=EDGE_CURVE ( 'NONE', #24765, #64553, #87665, .T. ) ;
#65960=FACE_OUTER_BOUND ( 'NONE', #112413, .T. ) ;
#65961=CARTESIAN_POINT ( 'NONE',  ( -11.64999999999999680, 12.50000000000000000, -2.792790559304612508 ) ) ;
#65962=ADVANCED_FACE ( 'NONE', ( #67357 ), #90351, .T. ) ;
#65963=VECTOR ( 'NONE', #99758, 1000.000000000000000 ) ;
#65964=DIRECTION ( 'NONE',  ( -0.000000000000000000, -1.000000000000000000, -0.000000000000000000 ) ) ;
#65965=VECTOR ( 'NONE', #34170, 1000.000000000000000 ) ;
#65967=ORIENTED_EDGE ( 'NONE', *, *, #19328, .T. ) ;
#65968=CIRCLE ( 'NONE', #55514, 0.06509327318403745899 ) ;
#65969=DIRECTION ( 'NONE',  ( -0.000000000000000000, 1.000000000000000000, -0.000000000000000000 ) ) ;
#65970=AXIS2_PLACEMENT_3D ( 'NONE', #43904, #105388, #33443 ) ;
#65971=ORIENTED_EDGE ( 'NONE', *, *, #79152, .F. ) ;
#65972=CARTESIAN_POINT ( 'NONE',  ( 21.15177371151418129, -2.593223176056361989, -4.151029080743455779 ) ) ;
#65973=DIRECTION ( 'NONE',  ( 0.000000000000000000, -0.9999939076577903929, 0.003490651415223739937 ) ) ;
#65974=PRODUCT_DEFINITION ( 'UNKNOWN', '', #113204, #6147 ) ;
#65975=FACE_OUTER_BOUND ( 'NONE', #124533, .T. ) ;
#65976=LINE ( 'NONE', #54231, #25539 ) ;
#65977=ORIENTED_EDGE ( 'NONE', *, *, #108255, .T. ) ;
#65978=ORIENTED_EDGE ( 'NONE', *, *, #20878, .F. ) ;
#65979=EDGE_LOOP ( 'NONE', ( #109148, #9704 ) ) ;
#65980=FACE_OUTER_BOUND ( 'NONE', #6831, .T. ) ;
#65981=CARTESIAN_POINT ( 'NONE',  ( 0.5999999999999612310, 2.500000000000000000, -0.4464101615137760493 ) ) ;
#65982=DIRECTION ( 'NONE',  ( 0.000000000000000000, -0.9999939076577903929, 0.003490651415223739937 ) ) ;
#65983=FACE_BOUND ( 'NONE', #42777, .T. ) ;
#65984=LINE ( 'NONE', #24783, #91146 ) ;
#65985=AXIS2_PLACEMENT_3D ( 'NONE', #12559, #53154, #4030 ) ;
#65986=CARTESIAN_POINT ( 'NONE',  ( -7.499999999999976907, 2.500000000000000000, 4.430127018922196847 ) ) ;
#65987=CARTESIAN_POINT ( 'NONE',  ( -12.29999999999999538, 12.50000000000000000, 4.611443907251934426 ) ) ;
#65988=CARTESIAN_POINT ( 'NONE',  ( -0.6500000000000403233, 2.500000000000000000, 1.818653347947321475 ) ) ;
#65990=AXIS2_PLACEMENT_3D ( 'NONE', #119800, #32086, #11773 ) ;
#65991=CARTESIAN_POINT ( 'NONE',  ( 14.99999999999989164, 12.50000000000000000, 0.7579135962115869374 ) ) ;
#65992=CARTESIAN_POINT ( 'NONE',  ( -8.350000000000012079, 12.50000000000000000, -2.857883832488653741 ) ) ;
#65993=CONICAL_SURFACE ( 'NONE', #38842, 0.09999999999999999167, 0.003490658503988666988 ) ;
#65994=CONICAL_SURFACE ( 'NONE', #51446, 0.09999999999999982514, 0.003490658503988666988 ) ;
#65995=DIRECTION ( 'NONE',  ( -0.000000000000000000, -1.000000000000000000, -0.000000000000000000 ) ) ;
#65996=AXIS2_PLACEMENT_3D ( 'NONE', #59081, #98997, #111374 ) ;
#65997=ORIENTED_EDGE ( 'NONE', *, *, #127903, .T. ) ;
#65998=B_SPLINE_CURVE_WITH_KNOTS ( 'NONE', 3,
 ( #102794, #94270, #103461, #13119, #22336, #93003, #4574, #104102 ),
 .UNSPECIFIED., .F., .F.,
 ( 4, 2, 2, 4 ),
 ( 0.000000000000000000, 0.01659259069806624451, 0.03318518139613248902, 0.06637036279226497804 ),
 .UNSPECIFIED. ) ;
#65999=ORIENTED_EDGE ( 'NONE', *, *, #37021, .F. ) ;
#66000=EDGE_LOOP ( 'NONE', ( #54684, #126974 ) ) ;
#66001=ORIENTED_EDGE ( 'NONE', *, *, #88687, .F. ) ;
#66002=DIRECTION ( 'NONE',  ( 0.000000000000000000, 1.000000000000000000, 0.000000000000000000 ) ) ;
#66003=EDGE_CURVE ( 'NONE', #38017, #1197, #98970, .T. ) ;
#66004=FACE_BOUND ( 'NONE', #39579, .T. ) ;
#66005=LINE ( 'NONE', #125561, #97488 ) ;
#66006=AXIS2_PLACEMENT_3D ( 'NONE', #123605, #1904, #44414 ) ;
#66007=EDGE_CURVE ( 'NONE', #22187, #119878, #44719, .T. ) ;
#66008=AXIS2_PLACEMENT_3D ( 'NONE', #124336, #52368, #92281 ) ;
#66009=AXIS2_PLACEMENT_3D ( 'NONE', #28526, #116879, #11288 ) ;
#66010=EDGE_CURVE ( 'NONE', #82094, #126222, #65448, .T. ) ;
#66011=ORIENTED_EDGE ( 'NONE', *, *, #121810, .T. ) ;
#66012=DIRECTION ( 'NONE',  ( 0.000000000000000000, 1.000000000000000000, 0.000000000000000000 ) ) ;
#66013=CARTESIAN_POINT ( 'NONE',  ( 8.749999999999918288, 2.500000000000000000, 7.188010851410848723 ) ) ;
#66014=VERTEX_POINT ( 'NONE', #107965 ) ;
#66015=DIRECTION ( 'NONE',  ( 0.000000000000000000, 0.000000000000000000, 1.000000000000000000 ) ) ;
#66016=DIRECTION ( 'NONE',  ( -0.000000000000000000, -1.000000000000000000, -0.000000000000000000 ) ) ;
#66017=ADVANCED_FACE ( 'NONE', ( #20876 ), #88286, .T. ) ;
#66018=CIRCLE ( 'NONE', #91064, 0.1000000000000002554 ) ;
#66019=CIRCLE ( 'NONE', #55563, 0.1000000000000002554 ) ;
#66020=VERTEX_POINT ( 'NONE', #59540 ) ;
#66021=DIRECTION ( 'NONE',  ( 0.000000000000000000, 1.000000000000000000, 0.000000000000000000 ) ) ;
#66022=DIRECTION ( 'NONE',  ( -0.000000000000000000, 1.000000000000000000, -0.000000000000000000 ) ) ;
#66023=ORIENTED_EDGE ( 'NONE', *, *, #117203, .T. ) ;
#66024=DIRECTION ( 'NONE',  ( 0.000000000000000000, 0.000000000000000000, -1.000000000000000000 ) ) ;
#66025=CARTESIAN_POINT ( 'NONE',  ( -4.150000000000028777, 2.500000000000000000, -5.802370205355749988 ) ) ;
#66026=ORIENTED_EDGE ( 'NONE', *, *, #29884, .F. ) ;
#66027=CARTESIAN_POINT ( 'NONE',  ( -0.2000000000000399791, 2.500000000000000000, -4.576537180435977348 ) ) ;
#66028=ORIENTED_EDGE ( 'NONE', *, *, #46756, .T. ) ;
#66029=ORIENTED_EDGE ( 'NONE', *, *, #89732, .F. ) ;
#66030=CARTESIAN_POINT ( 'NONE',  ( -10.00000000000000533, 2.500000000000000000, 5.022947341949748790 ) ) ;
#66031=EDGE_CURVE ( 'NONE', #60164, #67886, #60171, .T. ) ;
#66032=VERTEX_POINT ( 'NONE', #98778 ) ;
#66033=CARTESIAN_POINT ( 'NONE',  ( 7.499999999999925393, 2.500000000000000000, -0.6928203230275541413 ) ) ;
#66034=DIRECTION ( 'NONE',  ( 0.000000000000000000, 0.000000000000000000, -1.000000000000000000 ) ) ;
#66035=AXIS2_PLACEMENT_3D ( 'NONE', #50578, #41435, #81971 ) ;
#66036=ORIENTED_EDGE ( 'NONE', *, *, #76194, .F. ) ;
#66037=AXIS2_PLACEMENT_3D ( 'NONE', #109410, #102177, #102796 ) ;
#66039=DIRECTION ( 'NONE',  ( 0.000000000000000000, 0.000000000000000000, -1.000000000000000000 ) ) ;
#66041=DIRECTION ( 'NONE',  ( -0.000000000000000000, -1.000000000000000000, -0.000000000000000000 ) ) ;
#66042=PLANE ( 'NONE',  #77933 ) ;
#66043=CARTESIAN_POINT ( 'NONE',  ( 17.45053695044966346, 1.969637996572654481, -4.507340027902842827 ) ) ;
#66044=ORIENTED_EDGE ( 'NONE', *, *, #95664, .F. ) ;
#66045=EDGE_LOOP ( 'NONE', ( #100228, #103937, #439, #115737 ) ) ;
#66046=DIRECTION ( 'NONE',  ( 0.000000000000000000, 0.000000000000000000, 1.000000000000000000 ) ) ;
#66047=EDGE_CURVE ( 'NONE', #112495, #77768, #100081, .T. ) ;
#66048=FACE_OUTER_BOUND ( 'NONE', #26590, .T. ) ;
#66049=CARTESIAN_POINT ( 'NONE',  ( -3.550000000000027800, 12.50000000000000000, 6.083687093685482772 ) ) ;
#66050=AXIS2_PLACEMENT_3D ( 'NONE', #117439, #107664, #17982 ) ;
#66051=EDGE_LOOP ( 'NONE', ( #15912, #105020, #129088, #36642 ) ) ;
#66052=EDGE_LOOP ( 'NONE', ( #9811, #1856, #119629, #86644 ) ) ;
#66053=ORIENTED_EDGE ( 'NONE', *, *, #37474, .T. ) ;
#66054=FACE_OUTER_BOUND ( 'NONE', #10738, .T. ) ;
#66055=CARTESIAN_POINT ( 'NONE',  ( -2.500000000000031086, 2.500000000000000000, 3.637306695894644726 ) ) ;
#66056=CARTESIAN_POINT ( 'NONE',  ( 9.799999999999913669, 2.500000000000000000, 4.776537180435972196 ) ) ;
#66057=CONICAL_SURFACE ( 'NONE', #128785, 0.1000000000000000472, 0.003490658503988666988 ) ;
#66058=CARTESIAN_POINT ( 'NONE',  ( -11.64999999999999680, 12.50000000000000000, 7.188010851410848723 ) ) ;
#66059=CARTESIAN_POINT ( 'NONE',  ( -10.60000000000000320, 2.500000000000000000, -4.083716857408422385 ) ) ;
#66060=DIRECTION ( 'NONE',  ( -0.000000000000000000, -1.000000000000000000, -0.000000000000000000 ) ) ;
#66061=DIRECTION ( 'NONE',  ( 0.000000000000000000, 1.000000000000000000, 0.000000000000000000 ) ) ;
#66062=FACE_OUTER_BOUND ( 'NONE', #51264, .T. ) ;
#66063=EDGE_CURVE ( 'NONE', #79720, #37929, #38600, .T. ) ;
#66065=ORIENTED_EDGE ( 'NONE', *, *, #117958, .T. ) ;
#66066=DIRECTION ( 'NONE',  ( -0.000000000000000000, -1.000000000000000000, -0.000000000000000000 ) ) ;
#66067=EDGE_LOOP ( 'NONE', ( #129155, #81109, #85087, #12732 ) ) ;
#66068=EDGE_CURVE ( 'NONE', #55758, #30920, #13071, .T. ) ;
#66069=ORIENTED_EDGE ( 'NONE', *, *, #19097, .T. ) ;
#66070=DIRECTION ( 'NONE',  ( -0.000000000000000000, 1.000000000000000000, -0.000000000000000000 ) ) ;
#66071=CARTESIAN_POINT ( 'NONE',  ( 9.149999999999915090, 2.500000000000000000, -2.165063509461101710 ) ) ;
#66072=VECTOR ( 'NONE', #116407, 1000.000000000000000 ) ;
#66073=DIRECTION ( 'NONE',  ( -1.000000000000000000, 0.000000000000000000, -0.000000000000000000 ) ) ;
#66076=DIRECTION ( 'NONE',  ( 0.000000000000000000, 0.000000000000000000, -1.000000000000000000 ) ) ;
#66077=DIRECTION ( 'NONE',  ( 0.000000000000000000, 0.000000000000000000, -1.000000000000000000 ) ) ;
#66078=CONICAL_SURFACE ( 'NONE', #60137, 0.09999999999999982514, 0.003490658503988666988 ) ;
#66079=DIRECTION ( 'NONE',  ( 0.000000000000000000, 1.000000000000000000, 0.000000000000000000 ) ) ;
#66081=DIRECTION ( 'NONE',  ( 0.000000000000000000, 0.000000000000000000, 1.000000000000000000 ) ) ;
#66082=CIRCLE ( 'NONE', #110013, 0.06509327318403745899 ) ;
#66083=CIRCLE ( 'NONE', #74501, 0.1000000000000002554 ) ;
#66084=CARTESIAN_POINT ( 'NONE',  ( 0.1999999999999571565, 2.500000000000000000, 3.883716857408420431 ) ) ;
#66085=ORIENTED_EDGE ( 'NONE', *, *, #114967, .T. ) ;
#66086=ORIENTED_EDGE ( 'NONE', *, *, #117043, .T. ) ;
#66087=AXIS2_PLACEMENT_3D ( 'NONE', #87077, #85788, #127032 ) ;
#66088=ADVANCED_FACE ( 'NONE', ( #69308 ), #50335, .T. ) ;
#66089=ORIENTED_EDGE ( 'NONE', *, *, #18809, .F. ) ;
#66090=ORIENTED_EDGE ( 'NONE', *, *, #68939, .T. ) ;
#66091=CARTESIAN_POINT ( 'NONE',  ( -8.350000000000010303, 12.50000000000000000, 6.495190528383297135 ) ) ;
#66092=DIRECTION ( 'NONE',  ( 0.000000000000000000, -0.000000000000000000, 1.000000000000000000 ) ) ;
#66093=EDGE_CURVE ( 'NONE', #66296, #127206, #99448, .T. ) ;
#66094=DIRECTION ( 'NONE',  ( 0.000000000000000000, 0.000000000000000000, 1.000000000000000000 ) ) ;
#66095=DIRECTION ( 'NONE',  ( 0.000000000000000000, 1.000000000000000000, 0.000000000000000000 ) ) ;
#66096=AXIS2_PLACEMENT_3D ( 'NONE', #100789, #92936, #42557 ) ;
#66097=DIRECTION ( 'NONE',  ( 0.000000000000000000, 0.000000000000000000, -1.000000000000000000 ) ) ;
#66098=EDGE_LOOP ( 'NONE', ( #37922, #19089 ) ) ;
#66099=EDGE_CURVE ( 'NONE', #79663, #85834, #9116, .T. ) ;
#66100=ADVANCED_FACE ( 'NONE', ( #98134 ), #67432, .T. ) ;
#66101=EDGE_CURVE ( 'NONE', #71261, #122087, #90234, .T. ) ;
#66102=LINE ( 'NONE', #73342, #53535 ) ;
#66103=EDGE_CURVE ( 'NONE', #49433, #56692, #117613, .T. ) ;
#66104=DIRECTION ( 'NONE',  ( -0.000000000000000000, 1.000000000000000000, -0.000000000000000000 ) ) ;
#66105=VERTEX_POINT ( 'NONE', #18921 ) ;
#66106=VERTEX_POINT ( 'NONE', #50995 ) ;
#66107=EDGE_CURVE ( 'NONE', #35838, #78758, #107169, .T. ) ;
#66108=ORIENTED_EDGE ( 'NONE', *, *, #101917, .F. ) ;
#66109=DIRECTION ( 'NONE',  ( 0.000000000000000000, 0.000000000000000000, 1.000000000000000000 ) ) ;
#66110=ADVANCED_FACE ( 'NONE', ( #110536 ), #52798, .T. ) ;
#66112=DIRECTION ( 'NONE',  ( 0.000000000000000000, 1.000000000000000000, 0.000000000000000000 ) ) ;
#66113=DIRECTION ( 'NONE',  ( 0.000000000000000000, 0.000000000000000000, -1.000000000000000000 ) ) ;
#66114=EDGE_CURVE ( 'NONE', #55194, #90471, #123898, .T. ) ;
#66115=EDGE_CURVE ( 'NONE', #68282, #90560, #100707, .T. ) ;
#66116=ORIENTED_EDGE ( 'NONE', *, *, #19884, .T. ) ;
#66117=DIRECTION ( 'NONE',  ( -0.000000000000000000, -1.000000000000000000, -0.000000000000000000 ) ) ;
#66118=DIRECTION ( 'NONE',  ( 0.000000000000000000, 0.000000000000000000, -1.000000000000000000 ) ) ;
#66119=CARTESIAN_POINT ( 'NONE',  ( 12.69999999999990337, 2.500000000000000000, 3.983716857408420076 ) ) ;
#66120=DIRECTION ( 'NONE',  ( 0.000000000000000000, 0.000000000000000000, 1.000000000000000000 ) ) ;
#66121=CARTESIAN_POINT ( 'NONE',  ( -15.39999999999997904, 12.50000000000000000, 0.000000000000000000 ) ) ;
#66122=ADVANCED_FACE ( 'NONE', ( #30719 ), #90897, .T. ) ;
#66123=ORIENTED_EDGE ( 'NONE', *, *, #93173, .F. ) ;
#66124=CIRCLE ( 'NONE', #101652, 0.09999999999999982514 ) ;
#66125=DIRECTION ( 'NONE',  ( -0.000000000000000000, 1.000000000000000000, -0.000000000000000000 ) ) ;
#66126=AXIS2_PLACEMENT_3D ( 'NONE', #30727, #111165, #79794 ) ;
#66127=VERTEX_POINT ( 'NONE', #24097 ) ;
#66128=VERTEX_POINT ( 'NONE', #102012 ) ;
#66129=ORIENTED_EDGE ( 'NONE', *, *, #31221, .T. ) ;
#66130=DIRECTION ( 'NONE',  ( -0.000000000000000000, 1.000000000000000000, -0.000000000000000000 ) ) ;
#66131=FACE_BOUND ( 'NONE', #119604, .T. ) ;
#66132=DIRECTION ( 'NONE',  ( 0.000000000000000000, 0.000000000000000000, -1.000000000000000000 ) ) ;
#66134=CIRCLE ( 'NONE', #1383, 0.1000000000000000056 ) ;
#66135=AXIS2_PLACEMENT_3D ( 'NONE', #126864, #27341, #88187 ) ;
#66137=VERTEX_POINT ( 'NONE', #21520 ) ;
#66140=DIRECTION ( 'NONE',  ( 0.000000000000000000, 0.000000000000000000, 1.000000000000000000 ) ) ;
#66141=DIRECTION ( 'NONE',  ( -4.274815082592931898E-19, -0.9999939076577903929, -0.003490651415223739937 ) ) ;
#66142=EDGE_LOOP ( 'NONE', ( #102142, #79743 ) ) ;
#66143=CONICAL_SURFACE ( 'NONE', #80833, 0.1000000000000000472, 0.003490658503988666988 ) ;
#66144=AXIS2_PLACEMENT_3D ( 'NONE', #98333, #99643, #87223 ) ;
#66145=CARTESIAN_POINT ( 'NONE',  ( -3.300000000000027800, 2.500000000000000000, -4.430127018922202176 ) ) ;
#66146=VECTOR ( 'NONE', #53668, 1000.000000000000000 ) ;
#66147=DIRECTION ( 'NONE',  ( -4.274815082592931898E-19, -0.9999939076577903929, -0.003490651415223739937 ) ) ;
#66148=ORIENTED_EDGE ( 'NONE', *, *, #5948, .T. ) ;
#66149=CARTESIAN_POINT ( 'NONE',  ( -6.250000000000017764, 2.500000000000000000, 7.088010851410848190 ) ) ;
#66150=FACE_BOUND ( 'NONE', #36202, .T. ) ;
#66152=EDGE_CURVE ( 'NONE', #3902, #127429, #54844, .T. ) ;
#66153=ORIENTED_EDGE ( 'NONE', *, *, #97139, .T. ) ;
#66154=DIRECTION ( 'NONE',  ( 0.000000000000000000, 0.000000000000000000, 1.000000000000000000 ) ) ;
#66155=DIRECTION ( 'NONE',  ( -0.000000000000000000, 1.000000000000000000, -0.000000000000000000 ) ) ;
#66156=EDGE_CURVE ( 'NONE', #14509, #105930, #19340, .T. ) ;
#66157=ORIENTED_EDGE ( 'NONE', *, *, #19009, .F. ) ;
#66158=VERTEX_POINT ( 'NONE', #64019 ) ;
#66160=AXIS2_PLACEMENT_3D ( 'NONE', #1157, #60732, #100632 ) ;
#66161=VERTEX_POINT ( 'NONE', #12331 ) ;
#66163=CIRCLE ( 'NONE', #41163, 0.1000000000000002554 ) ;
#66164=DIRECTION ( 'NONE',  ( 0.000000000000000000, 1.000000000000000000, 0.000000000000000000 ) ) ;
#66165=ADVANCED_FACE ( 'NONE', ( #113112 ), #92179, .T. ) ;
#66166=AXIS2_PLACEMENT_3D ( 'NONE', #24610, #34443, #56618 ) ;
#66167=DIRECTION ( 'NONE',  ( -0.000000000000000000, -1.000000000000000000, -0.000000000000000000 ) ) ;
#66168=DIRECTION ( 'NONE',  ( 0.000000000000000000, 0.000000000000000000, -1.000000000000000000 ) ) ;
#66169=DIRECTION ( 'NONE',  ( -0.000000000000000000, -1.000000000000000000, -0.000000000000000000 ) ) ;
#66170=CONICAL_SURFACE ( 'NONE', #32762, 0.09999999999999982514, 0.003490658503988666988 ) ;
#66171=EDGE_LOOP ( 'NONE', ( #92989, #85688, #106781, #87805 ) ) ;
#66172=CONICAL_SURFACE ( 'NONE', #45261, 0.09999999999999982514, 0.003490658503988666988 ) ;
#66173=DIRECTION ( 'NONE',  ( 0.000000000000000000, -0.9999939076577903929, 0.003490651415223739937 ) ) ;
#66174=DIRECTION ( 'NONE',  ( 0.000000000000000000, -0.9999939076577903929, 0.003490651415223739937 ) ) ;
#66175=CARTESIAN_POINT ( 'NONE',  ( -10.65000000000000391, 2.500000000000000000, -1.718653347947322052 ) ) ;
#66176=CARTESIAN_POINT ( 'NONE',  ( -6.650000000000015454, 2.500000000000000000, 2.757883832488649656 ) ) ;
#66177=ORIENTED_EDGE ( 'NONE', *, *, #90672, .T. ) ;
#66178=ORIENTED_EDGE ( 'NONE', *, *, #83713, .T. ) ;
#66179=FACE_BOUND ( 'NONE', #38880, .T. ) ;
#66180=VERTEX_POINT ( 'NONE', #33914 ) ;
#66182=CARTESIAN_POINT ( 'NONE',  ( -11.89999999999999680, 2.500000000000000000, -0.2464101615137742063 ) ) ;
#66183=AXIS2_PLACEMENT_3D ( 'NONE', #1744, #90780, #1107 ) ;
#66184=ORIENTED_EDGE ( 'NONE', *, *, #74977, .F. ) ;
#66185=DIRECTION ( 'NONE',  ( 0.000000000000000000, 1.000000000000000000, 0.000000000000000000 ) ) ;
#66186=CARTESIAN_POINT ( 'NONE',  ( -3.550000000000031797, 2.500000000000000000, -6.248780366869526759 ) ) ;
#66187=FACE_OUTER_BOUND ( 'NONE', #119293, .T. ) ;
#66188=AXIS2_PLACEMENT_3D ( 'NONE', #107098, #77009, #114984 ) ;
#66189=DIRECTION ( 'NONE',  ( 0.000000000000000000, -0.9999939076577903929, 0.003490651415223739937 ) ) ;
#66190=ORIENTED_EDGE ( 'NONE', *, *, #91351, .T. ) ;
#66191=CARTESIAN_POINT ( 'NONE',  ( 13.54999999999990123, 2.500000000000000000, 1.918653347947321564 ) ) ;
#66192=DIRECTION ( 'NONE',  ( -0.000000000000000000, -1.000000000000000000, -0.000000000000000000 ) ) ;
#66194=CARTESIAN_POINT ( 'NONE',  ( -9.350000000000006750, 2.500000000000000000, -2.511473670974877948 ) ) ;
#66195=CARTESIAN_POINT ( 'NONE',  ( -12.49999999999999289, 2.500000000000000000, 3.537306695894645081 ) ) ;
#66196=ADVANCED_FACE ( 'NONE', ( #2497 ), #561, .T. ) ;
#66197=ORIENTED_EDGE ( 'NONE', *, *, #26127, .F. ) ;
#66198=VERTEX_POINT ( 'NONE', #42464 ) ;
#66199=DIRECTION ( 'NONE',  ( -4.274815082592931898E-19, -0.9999939076577903929, -0.003490651415223739937 ) ) ;
#66200=ORIENTED_EDGE ( 'NONE', *, *, #98594, .T. ) ;
#66201=CARTESIAN_POINT ( 'NONE',  ( -6.850000000000017408, 2.500000000000000000, -6.148780366869526226 ) ) ;
#66202=VERTEX_POINT ( 'NONE', #31354 ) ;
#66203=VERTEX_POINT ( 'NONE', #32656 ) ;
#66204=ORIENTED_EDGE ( 'NONE', *, *, #50573, .T. ) ;
#66205=DIRECTION ( 'NONE',  ( 0.000000000000000000, 1.000000000000000000, 0.000000000000000000 ) ) ;
#66206=DIRECTION ( 'NONE',  ( 0.000000000000000000, 0.000000000000000000, 1.000000000000000000 ) ) ;
#66207=DIRECTION ( 'NONE',  ( 0.000000000000000000, 0.000000000000000000, 1.000000000000000000 ) ) ;
#66209=FACE_OUTER_BOUND ( 'NONE', #55440, .T. ) ;
#66210=FACE_OUTER_BOUND ( 'NONE', #66984, .T. ) ;
#66211=EDGE_CURVE ( 'NONE', #126580, #31765, #21403, .T. ) ;
#66212=DIRECTION ( 'NONE',  ( 0.000000000000000000, 1.000000000000000000, 0.000000000000000000 ) ) ;
#66213=ORIENTED_EDGE ( 'NONE', *, *, #36405, .T. ) ;
#66214=EDGE_CURVE ( 'NONE', #65156, #121453, #65307, .T. ) ;
#66215=DIRECTION ( 'NONE',  ( -0.000000000000000000, -1.000000000000000000, -0.000000000000000000 ) ) ;
#66216=VERTEX_POINT ( 'NONE', #113771 ) ;
#66217=AXIS2_PLACEMENT_3D ( 'NONE', #106130, #6597, #47218 ) ;
#66218=EDGE_LOOP ( 'NONE', ( #28246, #62599, #81319, #118394 ) ) ;
#66219=ORIENTED_EDGE ( 'NONE', *, *, #37097, .F. ) ;
#66220=ORIENTED_EDGE ( 'NONE', *, *, #31293, .T. ) ;
#66221=CIRCLE ( 'NONE', #116387, 0.1000000000000002554 ) ;
#66222=CARTESIAN_POINT ( 'NONE',  ( -3.150000000000032330, 12.50000000000000000, -6.213873640053564351 ) ) ;
#66223=ORIENTED_EDGE ( 'NONE', *, *, #37055, .T. ) ;
#66224=ADVANCED_FACE ( 'NONE', ( #31997 ), #46525, .T. ) ;
#66225=ORIENTED_EDGE ( 'NONE', *, *, #4144, .T. ) ;
#66226=AXIS2_PLACEMENT_3D ( 'NONE', #10425, #60194, #39908 ) ;
#66227=AXIS2_PLACEMENT_3D ( 'NONE', #49288, #89191, #119944 ) ;
#66231=FACE_OUTER_BOUND ( 'NONE', #51259, .T. ) ;
#66232=FACE_OUTER_BOUND ( 'NONE', #45408, .T. ) ;
#66234=CIRCLE ( 'NONE', #72517, 0.06509327318403745899 ) ;
#66235=DIRECTION ( 'NONE',  ( 0.000000000000000000, 0.000000000000000000, 1.000000000000000000 ) ) ;
#66236=AXIS2_PLACEMENT_3D ( 'NONE', #113928, #64169, #124394 ) ;
#66237=AXIS2_PLACEMENT_3D ( 'NONE', #66783, #106710, #112540 ) ;
#66238=ORIENTED_EDGE ( 'NONE', *, *, #99955, .F. ) ;
#66239=CARTESIAN_POINT ( 'NONE',  ( -9.999999999999969802, 2.500000000000000000, -0.1000000000000022815 ) ) ;
#66240=AXIS2_PLACEMENT_3D ( 'NONE', #98362, #68261, #108828 ) ;
#66241=ORIENTED_EDGE ( 'NONE', *, *, #32799, .F. ) ;
#66242=DIRECTION ( 'NONE',  ( 0.000000000000000000, 1.000000000000000000, 0.000000000000000000 ) ) ;
#66243=ORIENTED_EDGE ( 'NONE', *, *, #100483, .T. ) ;
#66244=ORIENTED_EDGE ( 'NONE', *, *, #121635, .T. ) ;
#66245=CARTESIAN_POINT ( 'NONE',  ( 7.499999999999923617, 2.500000000000000000, 0.7928203230275495672 ) ) ;
#66246=DIRECTION ( 'NONE',  ( -4.274815082592931898E-19, -0.9999939076577903929, -0.003490651415223739937 ) ) ;
#66247=EDGE_CURVE ( 'NONE', #41822, #45891, #84183, .T. ) ;
#66248=DIRECTION ( 'NONE',  ( -0.000000000000000000, -1.000000000000000000, -0.000000000000000000 ) ) ;
#66249=CARTESIAN_POINT ( 'NONE',  ( -8.750000000000008882, 12.50000000000000000, -2.857883832488653741 ) ) ;
#66250=CARTESIAN_POINT ( 'NONE',  ( 8.749999999999921840, 2.500000000000000000, 2.957883832488649389 ) ) ;
#66251=ORIENTED_EDGE ( 'NONE', *, *, #108837, .F. ) ;
#66252=DIRECTION ( 'NONE',  ( -4.274815082592931898E-19, -0.9999939076577903929, -0.003490651415223739937 ) ) ;
#66253=DIRECTION ( 'NONE',  ( 0.000000000000000000, 0.000000000000000000, 1.000000000000000000 ) ) ;
#66254=ADVANCED_FACE ( 'NONE', ( #94122 ), #93486, .T. ) ;
#66255=DIRECTION ( 'NONE',  ( -0.000000000000000000, 1.000000000000000000, -0.000000000000000000 ) ) ;
#66256=CIRCLE ( 'NONE', #108020, 0.06509327318403745899 ) ;
#66257=CARTESIAN_POINT ( 'NONE',  ( 5.599999999999931255, 12.50000000000000000, 3.983716857408420076 ) ) ;
#66258=AXIS2_PLACEMENT_3D ( 'NONE', #33382, #93576, #81178 ) ;
#66259=EDGE_CURVE ( 'NONE', #87328, #37658, #94559, .T. ) ;
#66260=CONICAL_SURFACE ( 'NONE', #80943, 0.1000000000000002554, 0.003490658503988666988 ) ;
#66261=LINE ( 'NONE', #25691, #43813 ) ;
#66262=ORIENTED_EDGE ( 'NONE', *, *, #20241, .F. ) ;
#66263=AXIS2_PLACEMENT_3D ( 'NONE', #23156, #101731, #112840 ) ;
#66264=ORIENTED_EDGE ( 'NONE', *, *, #115428, .F. ) ;
#66266=EDGE_CURVE ( 'NONE', #71492, #34635, #23558, .T. ) ;
#66267=DIRECTION ( 'NONE',  ( 0.000000000000000000, -0.000000000000000000, 1.000000000000000000 ) ) ;
#66268=ADVANCED_FACE ( 'NONE', ( #61459 ), #101372, .T. ) ;
#66269=AXIS2_PLACEMENT_3D ( 'NONE', #46876, #85501, #86780 ) ;
#66270=ORIENTED_EDGE ( 'NONE', *, *, #10720, .T. ) ;
#66271=CIRCLE ( 'NONE', #80952, 0.06509327318403741736 ) ;
#66272=CARTESIAN_POINT ( 'NONE',  ( -2.500000000000030642, 2.500000000000000000, -5.022947341949754119 ) ) ;
#66273=DIRECTION ( 'NONE',  ( -0.000000000000000000, 1.000000000000000000, -0.000000000000000000 ) ) ;
#66274=CONICAL_SURFACE ( 'NONE', #51624, 0.1000000000000000472, 0.003490658503988666988 ) ;
#66275=ADVANCED_FACE ( 'NONE', ( #81714 ), #15115, .T. ) ;
#66276=ORIENTED_EDGE ( 'NONE', *, *, #14090, .T. ) ;
#66279=AXIS2_PLACEMENT_3D ( 'NONE', #65396, #35950, #85685 ) ;
#66280=FACE_OUTER_BOUND ( 'NONE', #86666, .T. ) ;
#66282=DIRECTION ( 'NONE',  ( 0.000000000000000000, 0.000000000000000000, -1.000000000000000000 ) ) ;
#66283=ORIENTED_EDGE ( 'NONE', *, *, #59152, .F. ) ;
#66284=ADVANCED_FACE ( 'NONE', ( #114397 ), #77837, .T. ) ;
#66285=CONICAL_SURFACE ( 'NONE', #118504, 0.1000000000000002554, 0.003490658503988666988 ) ;
#66286=CONICAL_SURFACE ( 'NONE', #97677, 0.1000000000000002554, 0.003490658503988666988 ) ;
#66287=CIRCLE ( 'NONE', #76667, 0.06509327318403745899 ) ;
#66288=CARTESIAN_POINT ( 'NONE',  ( -11.84999999999999609, 12.50000000000000000, 6.213873640053559022 ) ) ;
#66289=DIRECTION ( 'NONE',  ( 0.000000000000000000, -0.9999939076577903929, 0.003490651415223739937 ) ) ;
#66290=ORIENTED_EDGE ( 'NONE', *, *, #101124, .T. ) ;
#66291=DIRECTION ( 'NONE',  ( 0.000000000000000000, 0.000000000000000000, 1.000000000000000000 ) ) ;
#66292=DIRECTION ( 'NONE',  ( 0.000000000000000000, 0.000000000000000000, -1.000000000000000000 ) ) ;
#66293=DIRECTION ( 'NONE',  ( 0.000000000000000000, 0.000000000000000000, 1.000000000000000000 ) ) ;
#66294=ORIENTED_EDGE ( 'NONE', *, *, #105223, .T. ) ;
#66295=FACE_OUTER_BOUND ( 'NONE', #56201, .T. ) ;
#66296=VERTEX_POINT ( 'NONE', #96675 ) ;
#66297=CARTESIAN_POINT ( 'NONE',  ( -1.650000000000034328, 12.50000000000000000, -2.857883832488653741 ) ) ;
#66298=DIRECTION ( 'NONE',  ( -0.000000000000000000, -1.000000000000000000, -0.000000000000000000 ) ) ;
#66299=CIRCLE ( 'NONE', #41198, 0.06509327318403745899 ) ;
#66300=CARTESIAN_POINT ( 'NONE',  ( -12.49999999999995914, 12.50000000000000000, -4.395220292106237103 ) ) ;
#66301=ORIENTED_EDGE ( 'NONE', *, *, #41140, .F. ) ;
#66302=DIRECTION ( 'NONE',  ( 0.000000000000000000, 0.000000000000000000, 1.000000000000000000 ) ) ;
#66303=DIRECTION ( 'NONE',  ( -0.000000000000000000, -1.000000000000000000, -0.000000000000000000 ) ) ;
#66304=ORIENTED_EDGE ( 'NONE', *, *, #90935, .T. ) ;
#66305=EDGE_LOOP ( 'NONE', ( #120896, #13758, #104950, #65669 ) ) ;
#66306=FACE_OUTER_BOUND ( 'NONE', #124172, .T. ) ;
#66307=AXIS2_PLACEMENT_3D ( 'NONE', #29363, #120311, #30657 ) ;
#66308=EDGE_CURVE ( 'NONE', #5152, #32237, #56985, .T. ) ;
#66309=AXIS2_PLACEMENT_3D ( 'NONE', #1555, #41517, #42140 ) ;
#66310=ORIENTED_EDGE ( 'NONE', *, *, #1594, .F. ) ;
#66311=DIRECTION ( 'NONE',  ( 0.000000000000000000, 1.000000000000000000, 0.000000000000000000 ) ) ;
#66312=CARTESIAN_POINT ( 'NONE',  ( 6.649999999999930189, 12.50000000000000000, 5.867463478539781896 ) ) ;
#66313=ORIENTED_EDGE ( 'NONE', *, *, #67788, .T. ) ;
#66314=FACE_OUTER_BOUND ( 'NONE', #111035, .T. ) ;
#66315=CARTESIAN_POINT ( 'NONE',  ( -12.89999999999999325, 2.500000000000000000, -3.637306695894647390 ) ) ;
#66316=ORIENTED_EDGE ( 'NONE', *, *, #95695, .T. ) ;
#66317=AXIS2_PLACEMENT_3D ( 'NONE', #7028, #118938, #109099 ) ;
#66318=EDGE_CURVE ( 'NONE', #20664, #107019, #25592, .T. ) ;
#66319=DIRECTION ( 'NONE',  ( 0.000000000000000000, 0.000000000000000000, 1.000000000000000000 ) ) ;
#66320=DIRECTION ( 'NONE',  ( 0.000000000000000000, -0.9999939076577903929, 0.003490651415223739937 ) ) ;
#66321=AXIS2_PLACEMENT_3D ( 'NONE', #76690, #106777, #98251 ) ;
#66322=CARTESIAN_POINT ( 'NONE',  ( 4.599999999999938360, 12.50000000000000000, -2.276824562219559311E-15 ) ) ;
#66323=DIRECTION ( 'NONE',  ( 0.000000000000000000, 1.000000000000000000, 0.000000000000000000 ) ) ;
#66324=DIRECTION ( 'NONE',  ( 0.000000000000000000, 1.000000000000000000, 0.000000000000000000 ) ) ;
#66325=FACE_OUTER_BOUND ( 'NONE', #43388, .T. ) ;
#66327=AXIS2_PLACEMENT_3D ( 'NONE', #89666, #111212, #22874 ) ;
#66328=CONICAL_SURFACE ( 'NONE', #1576, 0.1000000000000002554, 0.003490658503988666988 ) ;
#66329=ORIENTED_EDGE ( 'NONE', *, *, #87920, .F. ) ;
#66330=ORIENTED_EDGE ( 'NONE', *, *, #86154, .T. ) ;
#66331=EDGE_LOOP ( 'NONE', ( #44648, #60391, #32679, #34841 ) ) ;
#66332=EDGE_LOOP ( 'NONE', ( #45199, #14154, #76696, #123468, #15780, #84507 ) ) ;
#66333=CARTESIAN_POINT ( 'NONE',  ( 6.649999999999930189, 2.500000000000000000, -2.957883832488653830 ) ) ;
#66334=CARTESIAN_POINT ( 'NONE',  ( 10.39999999999991509, 12.50000000000000000, 0.6928203230275494784 ) ) ;
#66335=DIRECTION ( 'NONE',  ( -4.274815082592931898E-19, -0.9999939076577903929, -0.003490651415223739937 ) ) ;
#66336=ORIENTED_EDGE ( 'NONE', *, *, #35735, .F. ) ;
#66337=FACE_BOUND ( 'NONE', #33733, .T. ) ;
#66338=DIRECTION ( 'NONE',  ( 0.000000000000000000, 1.000000000000000000, 0.000000000000000000 ) ) ;
#66339=DIRECTION ( 'NONE',  ( 0.000000000000000000, 1.000000000000000000, 0.000000000000000000 ) ) ;
#66340=CARTESIAN_POINT ( 'NONE',  ( -2.500000000000030642, 2.500000000000000000, -0.6928203230275541413 ) ) ;
#66341=DIRECTION ( 'NONE',  ( 0.000000000000000000, 0.000000000000000000, -1.000000000000000000 ) ) ;
#66342=DIRECTION ( 'NONE',  ( 0.000000000000000000, 1.000000000000000000, 0.000000000000000000 ) ) ;
#66343=VECTOR ( 'NONE', #48489, 1000.000000000000000 ) ;
#66344=CARTESIAN_POINT ( 'NONE',  ( -4.999999999999986677, 2.500000000000000000, -2.276824562219559311E-15 ) ) ;
#66345=DIRECTION ( 'NONE',  ( 0.000000000000000000, -0.9999939076577903929, 0.003490651415223739937 ) ) ;
#66346=CARTESIAN_POINT ( 'NONE',  ( 8.749999999999920064, 2.500000000000000000, 5.802370205355744659 ) ) ;
#66347=CARTESIAN_POINT ( 'NONE',  ( -12.04999999999999716, 2.500000000000000000, -2.165063509461097713 ) ) ;
#66348=AXIS2_PLACEMENT_3D ( 'NONE', #104367, #22125, #91478 ) ;
#66349=AXIS2_PLACEMENT_3D ( 'NONE', #118297, #9633, #68545 ) ;
#66350=PLANE ( 'NONE',  #77324 ) ;
#66351=EDGE_CURVE ( 'NONE', #41444, #128319, #90435, .T. ) ;
#66352=ORIENTED_EDGE ( 'NONE', *, *, #6545, .F. ) ;
#66353=CONICAL_SURFACE ( 'NONE', #11978, 0.09999999999999999167, 0.003490658503988666988 ) ;
#66354=ORIENTED_EDGE ( 'NONE', *, *, #61346, .T. ) ;
#66355=ORIENTED_EDGE ( 'NONE', *, *, #125512, .T. ) ;
#66356=EDGE_LOOP ( 'NONE', ( #63879, #128950 ) ) ;
#66357=CARTESIAN_POINT ( 'NONE',  ( -7.500000000000001776, 1.500000000000000000, -9.999999999999998224 ) ) ;
#66358=ORIENTED_EDGE ( 'NONE', *, *, #123422, .F. ) ;
#66359=DIRECTION ( 'NONE',  ( 0.000000000000000000, -0.9999939076577903929, 0.003490651415223739937 ) ) ;
#66360=ORIENTED_EDGE ( 'NONE', *, *, #101717, .T. ) ;
#66361=VERTEX_POINT ( 'NONE', #15542 ) ;
#66362=LINE ( 'NONE', #5497, #108572 ) ;
#66363=AXIS2_PLACEMENT_3D ( 'NONE', #19325, #79559, #80207 ) ;
#66364=EDGE_CURVE ( 'NONE', #87143, #19500, #23651, .T. ) ;
#66365=VECTOR ( 'NONE', #101018, 1000.000000000000000 ) ;
#66366=VECTOR ( 'NONE', #11715, 1000.000000000000000 ) ;
#66368=CARTESIAN_POINT ( 'NONE',  ( 1.249999999999953815, 12.50000000000000000, -2.857883832488653741 ) ) ;
#66369=CARTESIAN_POINT ( 'NONE',  ( -8.100000000000013856, 2.500000000000000000, 0.3464101615137736845 ) ) ;
#66370=DIRECTION ( 'NONE',  ( -0.000000000000000000, 1.000000000000000000, -0.000000000000000000 ) ) ;
#66371=CARTESIAN_POINT ( 'NONE',  ( 13.74999999999989875, 2.500000000000000000, 1.372243186433545370 ) ) ;
#66372=ADVANCED_FACE ( 'NONE', ( #36511 ), #92612, .T. ) ;
#66373=CONICAL_SURFACE ( 'NONE', #24523, 0.1000000000000002554, 0.003490658503988666988 ) ;
#66374=ADVANCED_FACE ( 'NONE', ( #46967 ), #65408, .T. ) ;
#66375=ORIENTED_EDGE ( 'NONE', *, *, #38047, .T. ) ;
#66376=ORIENTED_EDGE ( 'NONE', *, *, #76978, .T. ) ;
#66377=AXIS2_PLACEMENT_3D ( 'NONE', #17255, #106945, #118712 ) ;
#66378=CONICAL_SURFACE ( 'NONE', #53762, 0.09999999999999982514, 0.003490658503988666988 ) ;
#66379=VERTEX_POINT ( 'NONE', #55490 ) ;
#66380=VERTEX_POINT ( 'NONE', #75126 ) ;
#66381=EDGE_CURVE ( 'NONE', #40041, #119267, #88374, .T. ) ;
#66382=DIRECTION ( 'NONE',  ( 0.000000000000000000, 0.000000000000000000, 1.000000000000000000 ) ) ;
#66383=ORIENTED_EDGE ( 'NONE', *, *, #45695, .F. ) ;
#66384=EDGE_CURVE ( 'NONE', #96534, #44118, #7008, .T. ) ;
#66385=EDGE_LOOP ( 'NONE', ( #74919, #48662, #13893, #19794 ) ) ;
#66386=DIRECTION ( 'NONE',  ( 0.000000000000000000, 1.000000000000000000, 0.000000000000000000 ) ) ;
#66388=DIRECTION ( 'NONE',  ( 0.000000000000000000, 0.000000000000000000, -1.000000000000000000 ) ) ;
#66389=FACE_OUTER_BOUND ( 'NONE', #87224, .T. ) ;
#66390=DIRECTION ( 'NONE',  ( 0.000000000000000000, 1.000000000000000000, 0.000000000000000000 ) ) ;
#66391=DIRECTION ( 'NONE',  ( 0.000000000000000000, 0.000000000000000000, 1.000000000000000000 ) ) ;
#66392=ORIENTED_EDGE ( 'NONE', *, *, #86523, .T. ) ;
#66393=FACE_OUTER_BOUND ( 'NONE', #23513, .T. ) ;
#66394=ORIENTED_EDGE ( 'NONE', *, *, #87502, .T. ) ;
#66395=DIRECTION ( 'NONE',  ( 0.000000000000000000, 0.000000000000000000, 1.000000000000000000 ) ) ;
#66396=ORIENTED_EDGE ( 'NONE', *, *, #7943, .T. ) ;
#66397=DIRECTION ( 'NONE',  ( 0.000000000000000000, 1.000000000000000000, 0.000000000000000000 ) ) ;
#66398=FACE_OUTER_BOUND ( 'NONE', #19766, .T. ) ;
#66399=ORIENTED_EDGE ( 'NONE', *, *, #581, .T. ) ;
#66400=CARTESIAN_POINT ( 'NONE',  ( 4.349999999999940137, 2.500000000000000000, -2.511473670974877948 ) ) ;
#66401=DIRECTION ( 'NONE',  ( -0.000000000000000000, 1.000000000000000000, -0.000000000000000000 ) ) ;
#66402=ORIENTED_EDGE ( 'NONE', *, *, #63345, .T. ) ;
#66403=AXIS2_PLACEMENT_3D ( 'NONE', #84887, #62688, #124171 ) ;
#66404=EDGE_CURVE ( 'NONE', #44450, #129161, #98853, .T. ) ;
#66405=AXIS2_PLACEMENT_3D ( 'NONE', #28953, #69493, #28299 ) ;
#66406=CARTESIAN_POINT ( 'NONE',  ( -2.300000000000032685, 12.50000000000000000, -0.3464101615137783474 ) ) ;
#66407=ORIENTED_EDGE ( 'NONE', *, *, #20089, .T. ) ;
#66408=ORIENTED_EDGE ( 'NONE', *, *, #112879, .T. ) ;
#66409=FACE_OUTER_BOUND ( 'NONE', #18977, .T. ) ;
#66410=FACE_OUTER_BOUND ( 'NONE', #58342, .T. ) ;
#66413=CIRCLE ( 'NONE', #14168, 0.09999999999999999167 ) ;
#66414=EDGE_CURVE ( 'NONE', #27277, #56832, #8753, .T. ) ;
#66415=AXIS2_PLACEMENT_3D ( 'NONE', #87779, #58355, #38056 ) ;
#66416=CARTESIAN_POINT ( 'NONE',  ( 6.049999999999934097, 12.50000000000000000, 6.148780366869520897 ) ) ;
#66417=DIRECTION ( 'NONE',  ( -0.000000000000000000, -1.000000000000000000, -0.000000000000000000 ) ) ;
#66418=EDGE_CURVE ( 'NONE', #74873, #52167, #35851, .T. ) ;
#66419=EDGE_CURVE ( 'NONE', #103260, #6628, #36189, .T. ) ;
#66420=EDGE_CURVE ( 'NONE', #125657, #93435, #84941, .T. ) ;
#66421=ORIENTED_EDGE ( 'NONE', *, *, #69783, .T. ) ;
#66422=DIRECTION ( 'NONE',  ( -0.000000000000000000, 1.000000000000000000, -0.000000000000000000 ) ) ;
#66423=CIRCLE ( 'NONE', #3728, 0.1000000000000002554 ) ;
#66424=ORIENTED_EDGE ( 'NONE', *, *, #12454, .F. ) ;
#66425=EDGE_CURVE ( 'NONE', #45263, #125434, #86215, .T. ) ;
#66426=CONICAL_SURFACE ( 'NONE', #83173, 0.1000000000000002554, 0.003490658503988666988 ) ;
#66427=CARTESIAN_POINT ( 'NONE',  ( -4.076600168545496672E-14, 2.500000000000000000, -4.922947341949753586 ) ) ;
#66428=CARTESIAN_POINT ( 'NONE',  ( 9.799999999999918998, 12.50000000000000000, -0.3464101615137782364 ) ) ;
#66429=DIRECTION ( 'NONE',  ( -0.000000000000000000, -1.000000000000000000, -0.000000000000000000 ) ) ;
#66430=ORIENTED_EDGE ( 'NONE', *, *, #48525, .T. ) ;
#66431=ADVANCED_FACE ( 'NONE', ( #86870 ), #24740, .T. ) ;
#66432=CONICAL_SURFACE ( 'NONE', #33007, 0.1000000000000002554, 0.003490658503988666988 ) ;
#66433=EDGE_CURVE ( 'NONE', #45043, #32461, #111364, .T. ) ;
#66434=DIRECTION ( 'NONE',  ( 0.000000000000000000, 0.000000000000000000, 1.000000000000000000 ) ) ;
#66435=CARTESIAN_POINT ( 'NONE',  ( 7.949999999999922018, 2.500000000000000000, 6.495190528383297135 ) ) ;
#66436=VECTOR ( 'NONE', #59812, 1000.000000000000000 ) ;
#66437=AXIS2_PLACEMENT_3D ( 'NONE', #89877, #29048, #88597 ) ;
#66438=EDGE_LOOP ( 'NONE', ( #305, #116845, #29844, #33261 ) ) ;
#66439=AXIS2_PLACEMENT_3D ( 'NONE', #124348, #56233, #16922 ) ;
#66440=DIRECTION ( 'NONE',  ( 0.000000000000000000, 1.000000000000000000, 0.000000000000000000 ) ) ;
#66441=CIRCLE ( 'NONE', #114558, 0.06509327318403745899 ) ;
#66442=VERTEX_POINT ( 'NONE', #127455 ) ;
#66443=EDGE_LOOP ( 'NONE', ( #98854, #5079, #60929, #108035 ) ) ;
#66444=CARTESIAN_POINT ( 'NONE',  ( 3.099999999999943245, 2.500000000000000000, 3.983716857408420076 ) ) ;
#66445=AXIS2_PLACEMENT_3D ( 'NONE', #114799, #106278, #106908 ) ;
#66446=EDGE_LOOP ( 'NONE', ( #119505, #94394 ) ) ;
#66447=DIRECTION ( 'NONE',  ( -0.000000000000000000, 1.000000000000000000, -0.000000000000000000 ) ) ;
#66448=CARTESIAN_POINT ( 'NONE',  ( -11.64999999999999680, 12.50000000000000000, 1.537336459617582918 ) ) ;
#66449=CONICAL_SURFACE ( 'NONE', #83103, 0.1000000000000002554, 0.003490658503988666988 ) ;
#66450=DIRECTION ( 'NONE',  ( 0.000000000000000000, 1.000000000000000000, 0.000000000000000000 ) ) ;
#66451=ORIENTED_EDGE ( 'NONE', *, *, #81448, .F. ) ;
#66452=AXIS2_PLACEMENT_3D ( 'NONE', #75155, #42487, #104603 ) ;
#66453=FACE_BOUND ( 'NONE', #37258, .T. ) ;
#66454=DIRECTION ( 'NONE',  ( 0.000000000000000000, -0.9999939076577903929, 0.003490651415223739937 ) ) ;
#66455=VERTEX_POINT ( 'NONE', #8945 ) ;
#66456=LINE ( 'NONE', #16693, #102918 ) ;
#66457=CARTESIAN_POINT ( 'NONE',  ( 11.64999999999990443, 12.50000000000000000, 1.537336459617582918 ) ) ;
#66458=ORIENTED_EDGE ( 'NONE', *, *, #61067, .T. ) ;
#66459=CONICAL_SURFACE ( 'NONE', #124965, 0.09999999999999982514, 0.003490658503988666988 ) ;
#66460=CIRCLE ( 'NONE', #64322, 0.1000000000000002554 ) ;
#66461=EDGE_CURVE ( 'NONE', #11512, #45894, #50846, .T. ) ;
#66462=VERTEX_POINT ( 'NONE', #88135 ) ;
#66463=VERTEX_POINT ( 'NONE', #109068 ) ;
#66464=CARTESIAN_POINT ( 'NONE',  ( -6.050000000000017586, 12.50000000000000000, 6.148780366869520009 ) ) ;
#66465=PLANE ( 'NONE',  #93805 ) ;
#66466=DIRECTION ( 'NONE',  ( 0.000000000000000000, 1.000000000000000000, 0.000000000000000000 ) ) ;
#66467=FACE_BOUND ( 'NONE', #108462, .T. ) ;
#66468=EDGE_LOOP ( 'NONE', ( #49843, #36031 ) ) ;
#66470=CARTESIAN_POINT ( 'NONE',  ( 7.899999999999924860, 12.50000000000000000, -3.637306695894650055 ) ) ;
#66471=DIRECTION ( 'NONE',  ( 0.000000000000000000, -0.000000000000000000, 1.000000000000000000 ) ) ;
#66472=EDGE_CURVE ( 'NONE', #118333, #38253, #129416, .T. ) ;
#66473=FACE_OUTER_BOUND ( 'NONE', #125643, .T. ) ;
#66474=DIRECTION ( 'NONE',  ( -0.000000000000000000, -1.000000000000000000, -0.000000000000000000 ) ) ;
#66475=DIRECTION ( 'NONE',  ( 0.000000000000000000, 0.000000000000000000, 1.000000000000000000 ) ) ;
#66476=LINE ( 'NONE', #44256, #109823 ) ;
#66478=CARTESIAN_POINT ( 'NONE',  ( 1.049999999999954081, 12.50000000000000000, -6.148780366869526226 ) ) ;
#66479=ORIENTED_EDGE ( 'NONE', *, *, #127465, .T. ) ;
#66480=ORIENTED_EDGE ( 'NONE', *, *, #107143, .T. ) ;
#66481=EDGE_LOOP ( 'NONE', ( #42530, #64014, #108091, #41257 ) ) ;
#66482=AXIS2_PLACEMENT_3D ( 'NONE', #21614, #52354, #30807 ) ;
#66483=ORIENTED_EDGE ( 'NONE', *, *, #65948, .T. ) ;
#66484=ORIENTED_EDGE ( 'NONE', *, *, #115750, .T. ) ;
#66485=DIRECTION ( 'NONE',  ( 0.000000000000000000, 1.000000000000000000, 0.000000000000000000 ) ) ;
#66486=CIRCLE ( 'NONE', #10070, 0.06509327318403745899 ) ;
#66487=DIRECTION ( 'NONE',  ( 0.000000000000000000, 1.000000000000000000, 0.000000000000000000 ) ) ;
#66488=ORIENTED_EDGE ( 'NONE', *, *, #14346, .F. ) ;
#66489=FACE_BOUND ( 'NONE', #97997, .T. ) ;
#66490=CARTESIAN_POINT ( 'NONE',  ( 10.59999999999990905, 12.50000000000000000, 3.983716857408420076 ) ) ;
#66491=CIRCLE ( 'NONE', #62310, 0.09999999999999982514 ) ;
#66492=AXIS2_PLACEMENT_3D ( 'NONE', #81267, #83205, #92354 ) ;
#66494=DIRECTION ( 'NONE',  ( 0.000000000000000000, 0.000000000000000000, 1.000000000000000000 ) ) ;
#66495=FACE_OUTER_BOUND ( 'NONE', #40930, .T. ) ;
#66496=DIRECTION ( 'NONE',  ( -4.274815082592931898E-19, -0.9999939076577903929, -0.003490651415223739937 ) ) ;
#66497=ORIENTED_EDGE ( 'NONE', *, *, #24864, .T. ) ;
#66498=FACE_OUTER_BOUND ( 'NONE', #36676, .T. ) ;
#66499=CIRCLE ( 'NONE', #10082, 0.1000000000000002554 ) ;
#66500=B_SPLINE_CURVE_WITH_KNOTS ( 'NONE', 3,
 ( #49442, #78902, #20612, #71000, #69052, #19299, #101096, #48139 ),
 .UNSPECIFIED., .F., .F.,
 ( 4, 2, 2, 4 ),
 ( -1.045402497787284507E-05, 0.001241257413634800407, 0.001867113132941136070, 0.002492968852247471733 ),
 .UNSPECIFIED. ) ;
#66501=ORIENTED_EDGE ( 'NONE', *, *, #119489, .T. ) ;
#66502=EDGE_LOOP ( 'NONE', ( #53207, #53044, #77546, #108581 ) ) ;
#66503=ORIENTED_EDGE ( 'NONE', *, *, #52785, .F. ) ;
#66506=CARTESIAN_POINT ( 'NONE',  ( 4.149999999999936406, 2.500000000000000000, 6.595190528383296780 ) ) ;
#66507=ORIENTED_EDGE ( 'NONE', *, *, #79669, .T. ) ;
#66509=AXIS2_PLACEMENT_3D ( 'NONE', #127532, #107880, #27372 ) ;
#66510=ADVANCED_FACE ( 'NONE', ( #58711 ), #109324, .T. ) ;
#66512=DIRECTION ( 'NONE',  ( 0.000000000000000000, 1.000000000000000000, 0.000000000000000000 ) ) ;
#66514=DIRECTION ( 'NONE',  ( 0.000000000000000000, 1.000000000000000000, 0.000000000000000000 ) ) ;
#66515=EDGE_CURVE ( 'NONE', #87716, #93847, #80093, .T. ) ;
#66516=CARTESIAN_POINT ( 'NONE',  ( -4.250072516143177381E-14, 12.50000000000000000, -3.637306695894650055 ) ) ;
#66517=EDGE_CURVE ( 'NONE', #11592, #18164, #42453, .T. ) ;
#66518=VERTEX_POINT ( 'NONE', #40373 ) ;
#66519=CARTESIAN_POINT ( 'NONE',  ( -4.400000000000025224, 12.50000000000000000, -0.3464101615137783474 ) ) ;
#66520=CIRCLE ( 'NONE', #26827, 0.1000000000000002554 ) ;
#66521=VERTEX_POINT ( 'NONE', #37783 ) ;
#66522=VERTEX_POINT ( 'NONE', #77686 ) ;
#66524=DIRECTION ( 'NONE',  ( 0.000000000000000000, 0.000000000000000000, 1.000000000000000000 ) ) ;
#66525=EDGE_CURVE ( 'NONE', #37178, #17512, #110379, .T. ) ;
#66526=ADVANCED_FACE ( 'NONE', ( #109748 ), #27851, .T. ) ;
#66528=FACE_OUTER_BOUND ( 'NONE', #97471, .T. ) ;
#66529=ADVANCED_FACE ( 'NONE', ( #39740 ), #128117, .T. ) ;
#66530=ORIENTED_EDGE ( 'NONE', *, *, #49863, .F. ) ;
#66531=VECTOR ( 'NONE', #7777, 1000.000000000000000 ) ;
#66532=VERTEX_POINT ( 'NONE', #7658 ) ;
#66533=FACE_OUTER_BOUND ( 'NONE', #51208, .T. ) ;
#66534=CIRCLE ( 'NONE', #14299, 0.06509327318403743123 ) ;
#66535=FACE_OUTER_BOUND ( 'NONE', #26414, .T. ) ;
#66536=DIRECTION ( 'NONE',  ( 0.000000000000000000, 0.000000000000000000, 1.000000000000000000 ) ) ;
#66537=EDGE_LOOP ( 'NONE', ( #3165, #127989 ) ) ;
#66538=VERTEX_POINT ( 'NONE', #80292 ) ;
#66539=DIRECTION ( 'NONE',  ( 0.000000000000000000, 0.000000000000000000, 1.000000000000000000 ) ) ;
#66540=AXIS2_PLACEMENT_3D ( 'NONE', #101619, #42052, #102261 ) ;
#66541=ORIENTED_EDGE ( 'NONE', *, *, #21998, .F. ) ;
#66542=DIRECTION ( 'NONE',  ( -0.000000000000000000, 1.000000000000000000, -0.000000000000000000 ) ) ;
#66544=VERTEX_POINT ( 'NONE', #120211 ) ;
#66545=DIRECTION ( 'NONE',  ( 0.000000000000000000, 0.000000000000000000, -1.000000000000000000 ) ) ;
#66546=DIRECTION ( 'NONE',  ( 0.000000000000000000, 1.000000000000000000, 0.000000000000000000 ) ) ;
#66547=DIRECTION ( 'NONE',  ( -0.000000000000000000, -1.000000000000000000, -0.000000000000000000 ) ) ;
#66548=AXIS2_PLACEMENT_3D ( 'NONE', #4015, #52473, #113329 ) ;
#66549=CARTESIAN_POINT ( 'NONE',  ( 3.149999999999946176, 2.500000000000000000, -6.941600689897077459 ) ) ;
#66550=ORIENTED_EDGE ( 'NONE', *, *, #60918, .F. ) ;
#66551=CARTESIAN_POINT ( 'NONE',  ( 11.69999999999990870, 2.500000000000000000, 4.330127018922196314 ) ) ;
#66552=AXIS2_PLACEMENT_3D ( 'NONE', #13584, #112461, #22801 ) ;
#66553=CARTESIAN_POINT ( 'NONE',  ( -3.750000000000031086, 12.50000000000000000, -5.737276932171712751 ) ) ;
#66554=VERTEX_POINT ( 'NONE', #97982 ) ;
#66555=ORIENTED_EDGE ( 'NONE', *, *, #56637, .F. ) ;
#66557=DIRECTION ( 'NONE',  ( 0.000000000000000000, 0.000000000000000000, -1.000000000000000000 ) ) ;
#66558=CARTESIAN_POINT ( 'NONE',  ( 14.34999999999989662, 12.50000000000000000, 2.576566944158910744 ) ) ;
#66559=LINE ( 'NONE', #127436, #85614 ) ;
#66561=FACE_OUTER_BOUND ( 'NONE', #94450, .T. ) ;
#66562=CARTESIAN_POINT ( 'NONE',  ( 0.8499999999999536815, 12.50000000000000000, 5.802370205355744659 ) ) ;
#66563=DIRECTION ( 'NONE',  ( -0.000000000000000000, 1.000000000000000000, -0.000000000000000000 ) ) ;
#66564=LINE ( 'NONE', #76409, #2413 ) ;
#66565=EDGE_CURVE ( 'NONE', #94907, #82804, #54946, .T. ) ;
#66566=AXIS2_PLACEMENT_3D ( 'NONE', #110116, #139, #122516 ) ;
#66567=EDGE_CURVE ( 'NONE', #70903, #46827, #4755, .T. ) ;
#66568=ADVANCED_FACE ( 'NONE', ( #48906 ), #71678, .T. ) ;
#66569=DIRECTION ( 'NONE',  ( 0.000000000000000000, 1.000000000000000000, 0.000000000000000000 ) ) ;
#66570=VERTEX_POINT ( 'NONE', #99930 ) ;
#66571=AXIS2_PLACEMENT_3D ( 'NONE', #101531, #2660, #43910 ) ;
#66572=CONICAL_SURFACE ( 'NONE', #37353, 0.1000000000000002554, 0.003490658503988666988 ) ;
#66573=ORIENTED_EDGE ( 'NONE', *, *, #53719, .F. ) ;
#66574=CONICAL_SURFACE ( 'NONE', #70787, 0.09999999999999982514, 0.003490658503988666988 ) ;
#66575=CARTESIAN_POINT ( 'NONE',  ( 9.399999999999918643, 2.500000000000000000, 0.3464101615137736845 ) ) ;
#66576=EDGE_CURVE ( 'NONE', #84673, #76977, #31987, .T. ) ;
#66577=ORIENTED_EDGE ( 'NONE', *, *, #105381, .T. ) ;
#66578=EDGE_CURVE ( 'NONE', #122820, #23588, #69820, .T. ) ;
#66579=CARTESIAN_POINT ( 'NONE',  ( 14.14999999999989377, 2.500000000000000000, -2.857883832488653741 ) ) ;
#66580=DIRECTION ( 'NONE',  ( -0.000000000000000000, 1.000000000000000000, -0.000000000000000000 ) ) ;
#66581=CARTESIAN_POINT ( 'NONE',  ( 12.89999999999989910, 2.500000000000000000, 0.6928203230275494784 ) ) ;
#66582=CONICAL_SURFACE ( 'NONE', #129318, 0.1000000000000000472, 0.003490658503988666988 ) ;
#66583=EDGE_CURVE ( 'NONE', #47691, #90584, #117716, .T. ) ;
#66584=VERTEX_POINT ( 'NONE', #128765 ) ;
#66585=AXIS2_PLACEMENT_3D ( 'NONE', #81212, #80571, #82507 ) ;
#66586=EDGE_CURVE ( 'NONE', #40907, #56626, #113536, .T. ) ;
#66587=DIRECTION ( 'NONE',  ( 0.000000000000000000, 1.000000000000000000, 0.000000000000000000 ) ) ;
#66588=AXIS2_PLACEMENT_3D ( 'NONE', #114571, #75299, #124412 ) ;
#66589=ADVANCED_FACE ( 'NONE', ( #70461 ), #73824, .T. ) ;
#66590=CARTESIAN_POINT ( 'NONE',  ( -8.100000000000010303, 2.500000000000000000, 3.983716857408420964 ) ) ;
#66591=DIRECTION ( 'NONE',  ( -0.000000000000000000, -1.000000000000000000, -0.000000000000000000 ) ) ;
#66592=VERTEX_POINT ( 'NONE', #120848 ) ;
#66593=EDGE_CURVE ( 'NONE', #91689, #30841, #121844, .T. ) ;
#66594=CONICAL_SURFACE ( 'NONE', #10175, 0.09999999999999982514, 0.003490658503988666988 ) ;
#66595=CARTESIAN_POINT ( 'NONE',  ( -4.550000000000022915, 2.500000000000000000, -2.165063509461101710 ) ) ;
#66596=VERTEX_POINT ( 'NONE', #52746 ) ;
#66597=AXIS2_PLACEMENT_3D ( 'NONE', #54344, #46450, #126961 ) ;
#66598=ORIENTED_EDGE ( 'NONE', *, *, #126748, .T. ) ;
#66599=ORIENTED_EDGE ( 'NONE', *, *, #19811, .F. ) ;
#66600=EDGE_LOOP ( 'NONE', ( #124849, #720 ) ) ;
#66601=LINE ( 'NONE', #28627, #92901 ) ;
#66602=CARTESIAN_POINT ( 'NONE',  ( 1.049999999999952971, 2.500000000000000000, 6.148780366869520897 ) ) ;
#66603=DIRECTION ( 'NONE',  ( 0.000000000000000000, 0.000000000000000000, 1.000000000000000000 ) ) ;
#66604=DIRECTION ( 'NONE',  ( 0.000000000000000000, 0.000000000000000000, -1.000000000000000000 ) ) ;
#66605=CIRCLE ( 'NONE', #100069, 0.06509327318403745899 ) ;
#66606=ORIENTED_EDGE ( 'NONE', *, *, #44276, .F. ) ;
#66607=CARTESIAN_POINT ( 'NONE',  ( 6.649999999999929301, 12.50000000000000000, -2.165063509461101710 ) ) ;
#66608=ORIENTED_EDGE ( 'NONE', *, *, #104767, .T. ) ;
#66609=CIRCLE ( 'NONE', #14372, 0.06509327318403743123 ) ;
#66611=CARTESIAN_POINT ( 'NONE',  ( 5.199999999999931788, 2.500000000000000000, 4.676537180435972552 ) ) ;
#66613=DIRECTION ( 'NONE',  ( -4.274815082592931898E-19, -0.9999939076577903929, -0.003490651415223739937 ) ) ;
#66614=EDGE_LOOP ( 'NONE', ( #64362, #128599, #6225, #51285 ) ) ;
#66616=ORIENTED_EDGE ( 'NONE', *, *, #65033, .T. ) ;
#66617=ORIENTED_EDGE ( 'NONE', *, *, #120396, .F. ) ;
#66618=CARTESIAN_POINT ( 'NONE',  ( -7.700000000000010836, 2.500000000000000000, 3.983716857408420964 ) ) ;
#66619=DIRECTION ( 'NONE',  ( 0.000000000000000000, 1.000000000000000000, 0.000000000000000000 ) ) ;
#66620=CARTESIAN_POINT ( 'NONE',  ( 1.249999999999952482, 12.50000000000000000, -5.867463478539787225 ) ) ;
#66621=FACE_BOUND ( 'NONE', #14889, .T. ) ;
#66623=DIRECTION ( 'NONE',  ( 0.000000000000000000, 0.000000000000000000, 1.000000000000000000 ) ) ;
#66624=DIRECTION ( 'NONE',  ( -0.000000000000000000, 1.000000000000000000, -0.000000000000000000 ) ) ;
#66625=DIRECTION ( 'NONE',  ( -0.000000000000000000, -1.000000000000000000, -0.000000000000000000 ) ) ;
#66626=CIRCLE ( 'NONE', #83370, 0.06509327318403745899 ) ;
#66627=ADVANCED_FACE ( 'NONE', ( #2339 ), #69619, .T. ) ;
#66630=CARTESIAN_POINT ( 'NONE',  ( -13.34999999999999076, 2.500000000000000000, -1.572243186433547990 ) ) ;
#66631=CARTESIAN_POINT ( 'NONE',  ( 5.849999999999933920, 2.500000000000000000, 6.495190528383297135 ) ) ;
#66632=VECTOR ( 'NONE', #68186, 1000.000000000000000 ) ;
#66633=CONICAL_SURFACE ( 'NONE', #47883, 0.1000000000000000472, 0.003490658503988666988 ) ;
#66634=EDGE_LOOP ( 'NONE', ( #52673, #39069, #99095, #123288 ) ) ;
#66635=ORIENTED_EDGE ( 'NONE', *, *, #101145, .F. ) ;
#66636=ORIENTED_EDGE ( 'NONE', *, *, #3955, .T. ) ;
#66637=VERTEX_POINT ( 'NONE', #1708 ) ;
#66638=AXIS2_PLACEMENT_3D ( 'NONE', #59439, #100611, #10927 ) ;
#66639=CARTESIAN_POINT ( 'NONE',  ( -4.150000000000024336, 12.50000000000000000, 1.407149913249508000 ) ) ;
#66640=FACE_BOUND ( 'NONE', #12478, .T. ) ;
#66641=CARTESIAN_POINT ( 'NONE',  ( 13.09999999999989839, 12.50000000000000000, 0.3464101615137735735 ) ) ;
#66642=DIRECTION ( 'NONE',  ( -4.274815082592931898E-19, -0.9999939076577903929, -0.003490651415223739937 ) ) ;
#66643=AXIS2_PLACEMENT_3D ( 'NONE', #62117, #13634, #14897 ) ;
#66644=ORIENTED_EDGE ( 'NONE', *, *, #4002, .T. ) ;
#66645=FACE_OUTER_BOUND ( 'NONE', #99639, .T. ) ;
#66647=ORIENTED_EDGE ( 'NONE', *, *, #67117, .F. ) ;
#66648=CARTESIAN_POINT ( 'NONE',  ( -8.750000000000010658, 2.500000000000000000, 2.857883832488649301 ) ) ;
#66649=DIRECTION ( 'NONE',  ( 0.000000000000000000, 0.000000000000000000, 1.000000000000000000 ) ) ;
#66650=ORIENTED_EDGE ( 'NONE', *, *, #16335, .F. ) ;
#66651=CONICAL_SURFACE ( 'NONE', #1815, 0.1000000000000002554, 0.003490658503988666988 ) ;
#66652=DIRECTION ( 'NONE',  ( 0.000000000000000000, 1.000000000000000000, 0.000000000000000000 ) ) ;
#66653=FACE_OUTER_BOUND ( 'NONE', #120600, .T. ) ;
#66654=ORIENTED_EDGE ( 'NONE', *, *, #55185, .F. ) ;
#66655=AXIS2_PLACEMENT_3D ( 'NONE', #41829, #11042, #73206 ) ;
#66656=EDGE_CURVE ( 'NONE', #80887, #26124, #103071, .T. ) ;
#66657=LINE ( 'NONE', #38532, #113710 ) ;
#66658=AXIS2_PLACEMENT_3D ( 'NONE', #45818, #6485, #46440 ) ;
#66659=CARTESIAN_POINT ( 'NONE',  ( 5.199999999999935341, 12.50000000000000000, -0.3464101615137783474 ) ) ;
#66660=ORIENTED_EDGE ( 'NONE', *, *, #31802, .F. ) ;
#66661=DIRECTION ( 'NONE',  ( 0.000000000000000000, 0.000000000000000000, -1.000000000000000000 ) ) ;
#66662=ORIENTED_EDGE ( 'NONE', *, *, #114151, .T. ) ;
#66663=ORIENTED_EDGE ( 'NONE', *, *, #599, .T. ) ;
#66664=ADVANCED_FACE ( 'NONE', ( #92030 ), #90744, .T. ) ;
#66665=CARTESIAN_POINT ( 'NONE',  ( 0.6499999999999561684, 2.500000000000000000, -2.511473670974877948 ) ) ;
#66666=EDGE_CURVE ( 'NONE', #51434, #12584, #22665, .T. ) ;
#66667=ORIENTED_EDGE ( 'NONE', *, *, #51640, .F. ) ;
#66668=DIRECTION ( 'NONE',  ( 0.000000000000000000, 1.000000000000000000, 0.000000000000000000 ) ) ;
#66669=CARTESIAN_POINT ( 'NONE',  ( -2.100000000000034284, 12.50000000000000000, -2.385244779468109755E-15 ) ) ;
#66670=CONICAL_SURFACE ( 'NONE', #91725, 0.1000000000000002554, 0.003490658503988666988 ) ;
#66671=AXIS2_PLACEMENT_3D ( 'NONE', #94083, #105831, #95374 ) ;
#66672=ORIENTED_EDGE ( 'NONE', *, *, #46143, .T. ) ;
#66673=DIRECTION ( 'NONE',  ( 0.000000000000000000, -0.000000000000000000, 1.000000000000000000 ) ) ;
#66674=PLANE ( 'NONE',  #69162 ) ;
#66675=FACE_OUTER_BOUND ( 'NONE', #128058, .T. ) ;
#66676=EDGE_CURVE ( 'NONE', #54499, #49457, #115673, .T. ) ;
#66677=EDGE_CURVE ( 'NONE', #86613, #74320, #9073, .T. ) ;
#66678=DIRECTION ( 'NONE',  ( -0.000000000000000000, 1.000000000000000000, -0.000000000000000000 ) ) ;
#66679=EDGE_CURVE ( 'NONE', #41126, #61697, #94751, .T. ) ;
#66680=CARTESIAN_POINT ( 'NONE',  ( 10.84999999999990905, 2.500000000000000000, -5.902370205355750521 ) ) ;
#66681=EDGE_CURVE ( 'NONE', #96385, #3617, #21356, .T. ) ;
#66682=EDGE_CURVE ( 'NONE', #27458, #117981, #78137, .T. ) ;
#66683=CARTESIAN_POINT ( 'NONE',  ( 17.50000000000000355, 2.481874935395226078, -3.264429721014347585 ) ) ;
#66684=AXIS2_PLACEMENT_3D ( 'NONE', #70339, #110262, #70986 ) ;
#66685=ORIENTED_EDGE ( 'NONE', *, *, #49014, .F. ) ;
#66686=AXIS2_PLACEMENT_3D ( 'NONE', #21517, #82384, #122943 ) ;
#66687=ORIENTED_EDGE ( 'NONE', *, *, #46214, .T. ) ;
#66688=DIRECTION ( 'NONE',  ( 0.000000000000000000, 0.000000000000000000, 1.000000000000000000 ) ) ;
#66690=PLANE ( 'NONE',  #16711 ) ;
#66691=EDGE_LOOP ( 'NONE', ( #58892, #12819, #35413, #123106 ) ) ;
#66693=ORIENTED_EDGE ( 'NONE', *, *, #102018, .F. ) ;
#66694=EDGE_CURVE ( 'NONE', #77155, #31364, #122158, .T. ) ;
#66695=DIRECTION ( 'NONE',  ( -0.000000000000000000, -1.000000000000000000, -0.000000000000000000 ) ) ;
#66696=CARTESIAN_POINT ( 'NONE',  ( -14.99999999999994671, 12.50000000000000000, 0.000000000000000000 ) ) ;
#66697=ADVANCED_FACE ( 'NONE', ( #101215 ), #21699, .T. ) ;
#66698=LINE ( 'NONE', #66056, #49837 ) ;
#66699=DIRECTION ( 'NONE',  ( 0.000000000000000000, 1.000000000000000000, 0.000000000000000000 ) ) ;
#66701=DIRECTION ( 'NONE',  ( 0.000000000000000000, 0.000000000000000000, 1.000000000000000000 ) ) ;
#66702=CARTESIAN_POINT ( 'NONE',  ( -10.00000000000000533, 12.50000000000000000, 4.957854068765711553 ) ) ;
#66703=CONICAL_SURFACE ( 'NONE', #56240, 0.09999999999999982514, 0.003490658503988666988 ) ;
#66704=CARTESIAN_POINT ( 'NONE',  ( -12.09999999999999609, 12.50000000000000000, 0.6928203230275535862 ) ) ;
#66706=ORIENTED_EDGE ( 'NONE', *, *, #58420, .T. ) ;
#66707=DIRECTION ( 'NONE',  ( 0.000000000000000000, 0.000000000000000000, -1.000000000000000000 ) ) ;
#66709=ORIENTED_EDGE ( 'NONE', *, *, #70743, .T. ) ;
#66710=CARTESIAN_POINT ( 'NONE',  ( -9.350000000000008527, 2.500000000000000000, -6.941600689897073018 ) ) ;
#66711=CARTESIAN_POINT ( 'NONE',  ( 3.749999999999978684, 2.500000000000000000, -2.265063509461101798 ) ) ;
#66712=CONICAL_SURFACE ( 'NONE', #91868, 0.1000000000000002554, 0.003490658503988666988 ) ;
#66713=DIRECTION ( 'NONE',  ( -0.000000000000000000, 1.000000000000000000, -0.000000000000000000 ) ) ;
#66714=CARTESIAN_POINT ( 'NONE',  ( 7.699999999999922018, 2.500000000000000000, 0.2464101615137735679 ) ) ;
#66715=VECTOR ( 'NONE', #66454, 1000.000000000000000 ) ;
#66716=CARTESIAN_POINT ( 'NONE',  ( -4.150000000000027889, 2.500000000000000000, -6.395190528383301931 ) ) ;
#66717=LINE ( 'NONE', #48381, #120149 ) ;
#66718=DIRECTION ( 'NONE',  ( -0.000000000000000000, 1.000000000000000000, -0.000000000000000000 ) ) ;
#66720=CARTESIAN_POINT ( 'NONE',  ( 3.149999999999946176, 2.500000000000000000, -6.148780366869526226 ) ) ;
#66721=EDGE_CURVE ( 'NONE', #62965, #69394, #91384, .T. ) ;
#66722=EDGE_CURVE ( 'NONE', #27, #110433, #15316, .T. ) ;
#66723=DIRECTION ( 'NONE',  ( 0.000000000000000000, 1.000000000000000000, 0.000000000000000000 ) ) ;
#66724=ORIENTED_EDGE ( 'NONE', *, *, #5924, .F. ) ;
#66725=ORIENTED_EDGE ( 'NONE', *, *, #126969, .F. ) ;
#66726=EDGE_CURVE ( 'NONE', #92801, #125152, #59272, .T. ) ;
#66727=AXIS2_PLACEMENT_3D ( 'NONE', #48904, #126807, #69154 ) ;
#66728=AXIS2_PLACEMENT_3D ( 'NONE', #60698, #90783, #10297 ) ;
#66729=EDGE_LOOP ( 'NONE', ( #128461, #3463, #84765, #30422 ) ) ;
#66730=AXIS2_PLACEMENT_3D ( 'NONE', #43505, #4184, #83423 ) ;
#66731=ORIENTED_EDGE ( 'NONE', *, *, #67880, .F. ) ;
#66732=ADVANCED_FACE ( 'NONE', ( #119991 ), #18559, .T. ) ;
#66733=ORIENTED_EDGE ( 'NONE', *, *, #43422, .T. ) ;
#66734=LINE ( 'NONE', #106662, #115128 ) ;
#66735=CARTESIAN_POINT ( 'NONE',  ( 11.24999999999990941, 2.500000000000000000, -1.472243186433550122 ) ) ;
#66736=ADVANCED_FACE ( 'NONE', ( #119331 ), #751, .T. ) ;
#66737=AXIS2_PLACEMENT_3D ( 'NONE', #13590, #4395, #84921 ) ;
#66738=AXIS2_PLACEMENT_3D ( 'NONE', #79648, #59398, #1088 ) ;
#66739=EDGE_LOOP ( 'NONE', ( #70281, #105313 ) ) ;
#66741=DIRECTION ( 'NONE',  ( 0.000000000000000000, -0.9999939076577903929, 0.003490651415223739937 ) ) ;
#66742=EDGE_CURVE ( 'NONE', #113165, #1374, #80717, .T. ) ;
#66743=DIRECTION ( 'NONE',  ( 0.000000000000000000, 0.000000000000000000, -1.000000000000000000 ) ) ;
#66744=ORIENTED_EDGE ( 'NONE', *, *, #33492, .T. ) ;
#66745=DIRECTION ( 'NONE',  ( 0.000000000000000000, -0.9999939076577903929, 0.003490651415223739937 ) ) ;
#66746=ADVANCED_FACE ( 'NONE', ( #59811 ), #111474, .T. ) ;
#66747=DIRECTION ( 'NONE',  ( 0.000000000000000000, 0.000000000000000000, 1.000000000000000000 ) ) ;
#66748=ORIENTED_EDGE ( 'NONE', *, *, #55536, .F. ) ;
#66749=ORIENTED_EDGE ( 'NONE', *, *, #109980, .T. ) ;
#66750=ORIENTED_EDGE ( 'NONE', *, *, #129074, .F. ) ;
#66751=AXIS2_PLACEMENT_3D ( 'NONE', #117341, #59778, #47357 ) ;
#66752=DIRECTION ( 'NONE',  ( 0.000000000000000000, 0.000000000000000000, 1.000000000000000000 ) ) ;
#66753=CARTESIAN_POINT ( 'NONE',  ( 14.34999999999989662, 2.500000000000000000, 1.718653347947321386 ) ) ;
#66754=CIRCLE ( 'NONE', #33346, 0.06509327318403745899 ) ;
#66755=ORIENTED_EDGE ( 'NONE', *, *, #103819, .F. ) ;
#66756=DIRECTION ( 'NONE',  ( -0.000000000000000000, 1.000000000000000000, -0.000000000000000000 ) ) ;
#66757=DIRECTION ( 'NONE',  ( 0.000000000000000000, 0.000000000000000000, -1.000000000000000000 ) ) ;
#66758=DIRECTION ( 'NONE',  ( 0.000000000000000000, 0.000000000000000000, -1.000000000000000000 ) ) ;
#66760=EDGE_CURVE ( 'NONE', #121359, #5786, #2815, .T. ) ;
#66761=VECTOR ( 'NONE', #129087, 1000.000000000000000 ) ;
#66762=VECTOR ( 'NONE', #18096, 1000.000000000000000 ) ;
#66763=ORIENTED_EDGE ( 'NONE', *, *, #117779, .T. ) ;
#66764=CIRCLE ( 'NONE', #116934, 0.06509327318403745899 ) ;
#66765=DIRECTION ( 'NONE',  ( -0.000000000000000000, 1.000000000000000000, -0.000000000000000000 ) ) ;
#66766=EDGE_LOOP ( 'NONE', ( #113853, #108809 ) ) ;
#66767=VERTEX_POINT ( 'NONE', #118043 ) ;
#66768=ORIENTED_EDGE ( 'NONE', *, *, #46651, .T. ) ;
#66769=CARTESIAN_POINT ( 'NONE',  ( 12.09999999999990550, 12.50000000000000000, 4.395220292106234439 ) ) ;
#66770=FACE_BOUND ( 'NONE', #102776, .T. ) ;
#66771=DIRECTION ( 'NONE',  ( 0.000000000000000000, 0.000000000000000000, 1.000000000000000000 ) ) ;
#66772=CARTESIAN_POINT ( 'NONE',  ( -5.650000000000023448, 2.500000000000000000, -2.611473670974877592 ) ) ;
#66773=CARTESIAN_POINT ( 'NONE',  ( 3.749999999999942268, 2.500000000000000000, -5.802370205355749988 ) ) ;
#66774=VECTOR ( 'NONE', #118100, 1000.000000000000000 ) ;
#66775=ADVANCED_FACE ( 'NONE', ( #68947 ), #75967, .T. ) ;
#66776=ORIENTED_EDGE ( 'NONE', *, *, #100827, .T. ) ;
#66777=PLANE ( 'NONE',  #90246 ) ;
#66778=DIRECTION ( 'NONE',  ( 0.000000000000000000, -0.9999939076577903929, 0.003490651415223739937 ) ) ;
#66779=DIRECTION ( 'NONE',  ( 0.000000000000000000, 1.000000000000000000, 0.000000000000000000 ) ) ;
#66780=CARTESIAN_POINT ( 'NONE',  ( 7.099999999999926814, 2.500000000000000000, 0.09999999999999772959 ) ) ;
#66781=ORIENTED_EDGE ( 'NONE', *, *, #30492, .F. ) ;
#66782=CARTESIAN_POINT ( 'NONE',  ( -4.400000000000025224, 2.500000000000000000, 0.2464101615137735679 ) ) ;
#66783=CARTESIAN_POINT ( 'NONE',  ( 7.099999999999925926, 2.500000000000000000, 0.6928203230275494784 ) ) ;
#66784=CIRCLE ( 'NONE', #10370, 0.06509327318403745899 ) ;
#66785=ORIENTED_EDGE ( 'NONE', *, *, #97404, .T. ) ;
#66786=CARTESIAN_POINT ( 'NONE',  ( 14.14999999999989733, 2.500000000000000000, 1.472243186433545459 ) ) ;
#66787=ADVANCED_FACE ( 'NONE', ( #70889 ), #8714, .T. ) ;
#66788=DIRECTION ( 'NONE',  ( 0.000000000000000000, 0.000000000000000000, 1.000000000000000000 ) ) ;
#66789=FACE_BOUND ( 'NONE', #1158, .T. ) ;
#66790=CARTESIAN_POINT ( 'NONE',  ( 4.848431875627508880, -2.500000000000000000, -8.943854603337396014 ) ) ;
#66791=ORIENTED_EDGE ( 'NONE', *, *, #89902, .T. ) ;
#66792=DIRECTION ( 'NONE',  ( -0.000000000000000000, 1.000000000000000000, -0.000000000000000000 ) ) ;
#66793=ORIENTED_EDGE ( 'NONE', *, *, #7238, .F. ) ;
#66794=EDGE_LOOP ( 'NONE', ( #91556, #101992, #80441, #38555 ) ) ;
#66795=CARTESIAN_POINT ( 'NONE',  ( -1.010904742827955045E-17, 12.50000000000000000, -0.06509327318403743123 ) ) ;
#66797=EDGE_LOOP ( 'NONE', ( #126090, #31623 ) ) ;
#66798=CARTESIAN_POINT ( 'NONE',  ( 12.69999999999990337, 12.50000000000000000, 3.983716857408420076 ) ) ;
#66799=DIRECTION ( 'NONE',  ( 0.000000000000000000, 0.000000000000000000, -1.000000000000000000 ) ) ;
#66800=PLANE ( 'NONE',  #11347 ) ;
#66801=LINE ( 'NONE', #94335, #92383 ) ;
#66802=VECTOR ( 'NONE', #89237, 1000.000000000000000 ) ;
#66803=ORIENTED_EDGE ( 'NONE', *, *, #100529, .T. ) ;
#66804=EDGE_CURVE ( 'NONE', #86025, #34124, #71776, .T. ) ;
#66805=FACE_OUTER_BOUND ( 'NONE', #64745, .T. ) ;
#66806=CIRCLE ( 'NONE', #37600, 0.1000000000000002554 ) ;
#66807=CONICAL_SURFACE ( 'NONE', #6257, 0.1000000000000002554, 0.003490658503988666988 ) ;
#66808=CARTESIAN_POINT ( 'NONE',  ( 7.099999999999926814, 12.50000000000000000, -2.276824562219559311E-15 ) ) ;
#66809=DIRECTION ( 'NONE',  ( 0.000000000000000000, 0.000000000000000000, 1.000000000000000000 ) ) ;
#66810=DIRECTION ( 'NONE',  ( 0.000000000000000000, 0.000000000000000000, 1.000000000000000000 ) ) ;
#66811=VECTOR ( 'NONE', #48009, 1000.000000000000000 ) ;
#66812=ORIENTED_EDGE ( 'NONE', *, *, #58771, .F. ) ;
#66813=CARTESIAN_POINT ( 'NONE',  ( -2.499999999999996003, 12.50000000000000000, -0.06509327318403970719 ) ) ;
#66814=ORIENTED_EDGE ( 'NONE', *, *, #123340, .F. ) ;
#66815=CARTESIAN_POINT ( 'NONE',  ( 7.699999999999923794, 2.500000000000000000, -0.3464101615137783474 ) ) ;
#66816=DIRECTION ( 'NONE',  ( 0.000000000000000000, 0.000000000000000000, 1.000000000000000000 ) ) ;
#66817=ORIENTED_EDGE ( 'NONE', *, *, #45197, .T. ) ;
#66819=ADVANCED_FACE ( 'NONE', ( #10643 ), #70245, .T. ) ;
#66820=AXIS2_PLACEMENT_3D ( 'NONE', #51183, #20422, #91090 ) ;
#66821=CARTESIAN_POINT ( 'NONE',  ( -8.950000000000011724, 2.500000000000000000, -6.048780366869521252 ) ) ;
#66822=CARTESIAN_POINT ( 'NONE',  ( -10.84999999999999964, 2.500000000000000000, 7.188010851410848723 ) ) ;
#66823=CARTESIAN_POINT ( 'NONE',  ( 11.89999999999990443, 2.500000000000000000, 0.3464101615137736845 ) ) ;
#66824=ORIENTED_EDGE ( 'NONE', *, *, #66586, .F. ) ;
#66825=CARTESIAN_POINT ( 'NONE',  ( -10.45000000000000107, 2.500000000000000000, 6.495190528383297135 ) ) ;
#66826=FACE_OUTER_BOUND ( 'NONE', #13512, .T. ) ;
#66827=EDGE_CURVE ( 'NONE', #127840, #81996, #61058, .T. ) ;
#66828=EDGE_CURVE ( 'NONE', #128555, #26610, #96895, .T. ) ;
#66830=CARTESIAN_POINT ( 'NONE',  ( -2.100000000000034284, 2.500000000000000000, -2.385244779468109755E-15 ) ) ;
#66831=EDGE_CURVE ( 'NONE', #36298, #60265, #28391, .T. ) ;
#66832=ADVANCED_FACE ( 'NONE', ( #60446 ), #121950, .T. ) ;
#66833=DIRECTION ( 'NONE',  ( 0.000000000000000000, 0.000000000000000000, 1.000000000000000000 ) ) ;
#66834=ORIENTED_EDGE ( 'NONE', *, *, #60199, .F. ) ;
#66835=ORIENTED_EDGE ( 'NONE', *, *, #30980, .F. ) ;
#66837=EDGE_CURVE ( 'NONE', #88967, #43024, #40497, .T. ) ;
#66838=EDGE_LOOP ( 'NONE', ( #42046, #82664 ) ) ;
#66839=EDGE_CURVE ( 'NONE', #32739, #85461, #29043, .T. ) ;
#66840=CARTESIAN_POINT ( 'NONE',  ( 7.299999999999926104, 12.50000000000000000, -0.4115034346978156399 ) ) ;
#66841=ORIENTED_EDGE ( 'NONE', *, *, #27594, .T. ) ;
#66842=ORIENTED_EDGE ( 'NONE', *, *, #129402, .T. ) ;
#66843=ORIENTED_EDGE ( 'NONE', *, *, #76299, .T. ) ;
#66844=EDGE_CURVE ( 'NONE', #16096, #121037, #36289, .T. ) ;
#66845=FACE_OUTER_BOUND ( 'NONE', #26421, .T. ) ;
#66846=ADVANCED_FACE ( 'NONE', ( #129194 ), #29672, .T. ) ;
#66847=AXIS2_PLACEMENT_3D ( 'NONE', #31676, #59224, #31056 ) ;
#66848=DIRECTION ( 'NONE',  ( 0.000000000000000000, 0.000000000000000000, 1.000000000000000000 ) ) ;
#66849=EDGE_CURVE ( 'NONE', #34783, #42431, #119890, .T. ) ;
#66850=CONICAL_SURFACE ( 'NONE', #127413, 0.1000000000000000472, 0.003490658503988666988 ) ;
#66851=CARTESIAN_POINT ( 'NONE',  ( -11.64999999999999858, 12.50000000000000000, -5.802370205355746435 ) ) ;
#66853=CARTESIAN_POINT ( 'NONE',  ( -10.85000000000000142, 12.50000000000000000, -2.792790559304612508 ) ) ;
#66854=LINE ( 'NONE', #55751, #16668 ) ;
#66855=DIRECTION ( 'NONE',  ( 0.000000000000000000, 1.000000000000000000, 0.000000000000000000 ) ) ;
#66856=ORIENTED_EDGE ( 'NONE', *, *, #53439, .F. ) ;
#66857=EDGE_CURVE ( 'NONE', #111968, #74697, #86427, .T. ) ;
#66858=AXIS2_PLACEMENT_3D ( 'NONE', #102468, #52719, #63189 ) ;
#66859=CARTESIAN_POINT ( 'NONE',  ( 9.149999999999920419, 12.50000000000000000, 1.472243186433545459 ) ) ;
#66860=AXIS2_PLACEMENT_3D ( 'NONE', #60298, #100200, #40658 ) ;
#66861=ORIENTED_EDGE ( 'NONE', *, *, #127484, .F. ) ;
#66863=VERTEX_POINT ( 'NONE', #31612 ) ;
#66864=ORIENTED_EDGE ( 'NONE', *, *, #81644, .F. ) ;
#66865=CARTESIAN_POINT ( 'NONE',  ( -5.400000000000019895, 12.50000000000000000, 0.06509327318403515528 ) ) ;
#66866=ORIENTED_EDGE ( 'NONE', *, *, #58369, .F. ) ;
#66867=VERTEX_POINT ( 'NONE', #52534 ) ;
#66868=AXIS2_PLACEMENT_3D ( 'NONE', #122841, #20777, #91442 ) ;
#66869=AXIS2_PLACEMENT_3D ( 'NONE', #95743, #106207, #76100 ) ;
#66870=DIRECTION ( 'NONE',  ( 0.000000000000000000, 1.000000000000000000, 0.000000000000000000 ) ) ;
#66871=DIRECTION ( 'NONE',  ( -4.274815082592931898E-19, -0.9999939076577903929, -0.003490651415223739937 ) ) ;
#66872=CONICAL_SURFACE ( 'NONE', #75282, 0.1000000000000000472, 0.003490658503988666988 ) ;
#66873=DIRECTION ( 'NONE',  ( 0.000000000000000000, 0.000000000000000000, -1.000000000000000000 ) ) ;
#66874=DIRECTION ( 'NONE',  ( 0.000000000000000000, 0.000000000000000000, 1.000000000000000000 ) ) ;
#66875=LINE ( 'NONE', #117243, #30030 ) ;
#66876=ORIENTED_EDGE ( 'NONE', *, *, #26082, .F. ) ;
#66877=VECTOR ( 'NONE', #28213, 1000.000000000000000 ) ;
#66878=FACE_OUTER_BOUND ( 'NONE', #119021, .T. ) ;
#66879=AXIS2_PLACEMENT_3D ( 'NONE', #47150, #115879, #16993 ) ;
#66880=ORIENTED_EDGE ( 'NONE', *, *, #14144, .T. ) ;
#66881=LINE ( 'NONE', #17107, #4585 ) ;
#66882=ORIENTED_EDGE ( 'NONE', *, *, #67449, .F. ) ;
#66883=DIRECTION ( 'NONE',  ( 0.000000000000000000, -0.9999939076577903929, 0.003490651415223739937 ) ) ;
#66884=CIRCLE ( 'NONE', #71096, 0.1000000000000000472 ) ;
#66885=EDGE_LOOP ( 'NONE', ( #57842, #10949 ) ) ;
#66886=VERTEX_POINT ( 'NONE', #71520 ) ;
#66887=CARTESIAN_POINT ( 'NONE',  ( -8.150000000000009237, 12.50000000000000000, 6.776507416713035248 ) ) ;
#66888=LINE ( 'NONE', #115996, #102816 ) ;
#66889=ADVANCED_FACE ( 'NONE', ( #123833 ), #64281, .T. ) ;
#66891=CARTESIAN_POINT ( 'NONE',  ( -3.150000000000033218, 2.500000000000000000, -6.941600689897078347 ) ) ;
#66892=EDGE_CURVE ( 'NONE', #33146, #92869, #23757, .T. ) ;
#66893=DIRECTION ( 'NONE',  ( 0.000000000000000000, 1.000000000000000000, 0.000000000000000000 ) ) ;
#66894=ORIENTED_EDGE ( 'NONE', *, *, #113188, .T. ) ;
#66895=DIRECTION ( 'NONE',  ( 0.000000000000000000, 0.000000000000000000, 1.000000000000000000 ) ) ;
#66896=CARTESIAN_POINT ( 'NONE',  ( 8.749999999999957367, 12.50000000000000000, 2.165063509461097713 ) ) ;
#66897=FACE_OUTER_BOUND ( 'NONE', #80436, .T. ) ;
#66898=FACE_OUTER_BOUND ( 'NONE', #624, .T. ) ;
#66899=EDGE_CURVE ( 'NONE', #96815, #12366, #43380, .T. ) ;
#66900=DIRECTION ( 'NONE',  ( -4.274815082592931898E-19, -0.9999939076577903929, -0.003490651415223739937 ) ) ;
#66901=ORIENTED_EDGE ( 'NONE', *, *, #84425, .F. ) ;
#66902=ORIENTED_EDGE ( 'NONE', *, *, #72394, .F. ) ;
#66903=CARTESIAN_POINT ( 'NONE',  ( -8.950000000000004619, 2.500000000000000000, 6.048780366869521252 ) ) ;
#66904=VECTOR ( 'NONE', #7118, 1000.000000000000000 ) ;
#66905=VERTEX_POINT ( 'NONE', #42748 ) ;
#66906=DIRECTION ( 'NONE',  ( -0.000000000000000000, -1.000000000000000000, -0.000000000000000000 ) ) ;
#66907=CARTESIAN_POINT ( 'NONE',  ( -6.650000000000015454, 12.50000000000000000, 2.857883832488649301 ) ) ;
#66908=ORIENTED_EDGE ( 'NONE', *, *, #82930, .F. ) ;
#66910=DIRECTION ( 'NONE',  ( -0.000000000000000000, -1.000000000000000000, -0.000000000000000000 ) ) ;
#66911=CARTESIAN_POINT ( 'NONE',  ( 9.999999999999952038, 12.50000000000000000, -2.276824562219559311E-15 ) ) ;
#66913=CARTESIAN_POINT ( 'NONE',  ( 4.149999999999941735, 12.50000000000000000, -1.537336459617587581 ) ) ;
#66914=EDGE_LOOP ( 'NONE', ( #123965, #4924 ) ) ;
#66915=AXIS2_PLACEMENT_3D ( 'NONE', #32965, #122616, #123883 ) ;
#66916=FACE_OUTER_BOUND ( 'NONE', #32908, .T. ) ;
#66917=DIRECTION ( 'NONE',  ( 0.000000000000000000, 1.000000000000000000, 0.000000000000000000 ) ) ;
#66918=ORIENTED_EDGE ( 'NONE', *, *, #109262, .F. ) ;
#66919=DIRECTION ( 'NONE',  ( 0.000000000000000000, 0.000000000000000000, 1.000000000000000000 ) ) ;
#66920=DIRECTION ( 'NONE',  ( 0.000000000000000000, 0.000000000000000000, -1.000000000000000000 ) ) ;
#66921=DIRECTION ( 'NONE',  ( -0.000000000000000000, -1.000000000000000000, -0.000000000000000000 ) ) ;
#66922=EDGE_LOOP ( 'NONE', ( #98527, #90610 ) ) ;
#66923=DIRECTION ( 'NONE',  ( -4.274815082592931898E-19, -0.9999939076577903929, -0.003490651415223739937 ) ) ;
#66924=ORIENTED_EDGE ( 'NONE', *, *, #80025, .T. ) ;
#66925=FACE_OUTER_BOUND ( 'NONE', #60025, .T. ) ;
#66926=DIRECTION ( 'NONE',  ( 0.000000000000000000, -0.000000000000000000, 1.000000000000000000 ) ) ;
#66927=DIRECTION ( 'NONE',  ( 0.000000000000000000, 0.000000000000000000, 1.000000000000000000 ) ) ;
#66928=EDGE_LOOP ( 'NONE', ( #82242, #12385 ) ) ;
#66929=AXIS2_PLACEMENT_3D ( 'NONE', #55602, #44488, #24855 ) ;
#66930=DIRECTION ( 'NONE',  ( 0.000000000000000000, 0.000000000000000000, -1.000000000000000000 ) ) ;
#66931=CONICAL_SURFACE ( 'NONE', #43975, 0.1000000000000000472, 0.003490658503988666988 ) ;
#66932=DIRECTION ( 'NONE',  ( -0.000000000000000000, 1.000000000000000000, -0.000000000000000000 ) ) ;
#66933=EDGE_CURVE ( 'NONE', #57940, #10654, #34231, .T. ) ;
#66934=EDGE_LOOP ( 'NONE', ( #75163, #117277, #87163, #97980 ) ) ;
#66935=DIRECTION ( 'NONE',  ( 0.000000000000000000, 0.000000000000000000, 1.000000000000000000 ) ) ;
#66936=EDGE_CURVE ( 'NONE', #62733, #594, #34195, .T. ) ;
#66937=ORIENTED_EDGE ( 'NONE', *, *, #116034, .T. ) ;
#66938=DIRECTION ( 'NONE',  ( 0.000000000000000000, 1.000000000000000000, 0.000000000000000000 ) ) ;
#66939=ORIENTED_EDGE ( 'NONE', *, *, #32448, .T. ) ;
#66940=DIRECTION ( 'NONE',  ( 0.000000000000000000, 0.000000000000000000, 1.000000000000000000 ) ) ;
#66941=CARTESIAN_POINT ( 'NONE',  ( 7.699999999999923794, 12.50000000000000000, 4.676537180435972552 ) ) ;
#66942=ORIENTED_EDGE ( 'NONE', *, *, #17277, .T. ) ;
#66943=EDGE_CURVE ( 'NONE', #80214, #96136, #124087, .T. ) ;
#66944=VERTEX_POINT ( 'NONE', #53194 ) ;
#66945=DIRECTION ( 'NONE',  ( -0.000000000000000000, 1.000000000000000000, -0.000000000000000000 ) ) ;
#66946=CARTESIAN_POINT ( 'NONE',  ( 5.849999999999933920, 12.50000000000000000, 5.867463478539781896 ) ) ;
#66947=EDGE_LOOP ( 'NONE', ( #72269, #107320 ) ) ;
#66948=AXIS2_PLACEMENT_3D ( 'NONE', #32818, #21697, #83199 ) ;
#66949=FACE_OUTER_BOUND ( 'NONE', #86391, .T. ) ;
#66950=DIRECTION ( 'NONE',  ( 0.000000000000000000, 1.000000000000000000, 0.000000000000000000 ) ) ;
#66951=AXIS2_PLACEMENT_3D ( 'NONE', #79045, #28653, #118948 ) ;
#66952=FACE_OUTER_BOUND ( 'NONE', #114677, .T. ) ;
#66953=CARTESIAN_POINT ( 'NONE',  ( -0.6500000000000389910, 2.500000000000000000, -1.818653347947326138 ) ) ;
#66954=LINE ( 'NONE', #8674, #101697 ) ;
#66955=FACE_OUTER_BOUND ( 'NONE', #39435, .T. ) ;
#66956=AXIS2_PLACEMENT_3D ( 'NONE', #119743, #610, #77877 ) ;
#66957=ORIENTED_EDGE ( 'NONE', *, *, #14699, .F. ) ;
#66958=ADVANCED_FACE ( 'NONE', ( #114037 ), #62369, .T. ) ;
#66959=EDGE_LOOP ( 'NONE', ( #30903, #70646, #79611, #91739 ) ) ;
#66960=ORIENTED_EDGE ( 'NONE', *, *, #34003, .T. ) ;
#66963=DIRECTION ( 'NONE',  ( 0.000000000000000000, 0.000000000000000000, 1.000000000000000000 ) ) ;
#66964=DIRECTION ( 'NONE',  ( 0.000000000000000000, 1.000000000000000000, 0.000000000000000000 ) ) ;
#66965=CARTESIAN_POINT ( 'NONE',  ( -11.64999999999999680, 12.50000000000000000, -2.165063509461097713 ) ) ;
#66966=VERTEX_POINT ( 'NONE', #2138 ) ;
#66967=FACE_BOUND ( 'NONE', #15282, .T. ) ;
#66968=DIRECTION ( 'NONE',  ( 0.000000000000000000, 0.000000000000000000, 1.000000000000000000 ) ) ;
#66969=CARTESIAN_POINT ( 'NONE',  ( 12.29999999999990656, 2.500000000000000000, 3.883716857408421319 ) ) ;
#66970=FACE_OUTER_BOUND ( 'NONE', #121430, .T. ) ;
#66971=ADVANCED_FACE ( 'NONE', ( #2785 ), #81985, .T. ) ;
#66972=DIRECTION ( 'NONE',  ( 0.000000000000000000, 0.000000000000000000, 1.000000000000000000 ) ) ;
#66973=DIRECTION ( 'NONE',  ( 0.000000000000000000, -0.000000000000000000, 1.000000000000000000 ) ) ;
#66974=DIRECTION ( 'NONE',  ( 0.000000000000000000, 0.000000000000000000, -1.000000000000000000 ) ) ;
#66975=( BOUNDED_SURFACE ( )  B_SPLINE_SURFACE ( 3, 2, ( 
 ( #1086, #20735, #51495 ),
 ( #52134, #92043, #1722 ),
 ( #81579, #60672, #50208 ),
 ( #32512, #109091, #2349 ),
 ( #42313, #99301, #90095 ),
 ( #40388, #80308, #120227 ),
 ( #30574, #100568, #62603 ),
 ( #124728, #73059, #15401 ),
 ( #53426, #3666, #114261 ),
 ( #55349, #43611, #12815 ),
 ( #74341, #34436, #33766 ),
 ( #123434, #93341, #83530 ),
 ( #73685, #64512, #14744 ),
 ( #44226, #113624, #23958 ) ),
 .UNSPECIFIED., .F., .F., .F. ) 
 B_SPLINE_SURFACE_WITH_KNOTS ( ( 4, 2, 2, 2, 2, 2, 4 ),
 ( 3, 3 ),
 ( 0.000000000000000000, 0.001744612550434268029, 0.002616918825651402044, 0.003489225100868536059, 0.005233837651302804088, 0.006106143926519938536, 0.006978450201737072117 ),
 ( 0.000000000000000000, 1.000000000000000000 ),
 .UNSPECIFIED. ) 
 GEOMETRIC_REPRESENTATION_ITEM ( )  RATIONAL_B_SPLINE_SURFACE ( (
 ( 1.000000000000000000, 0.7318752858502209913, 1.000000000000000000),
 ( 1.000000000000000000, 0.7270130115579832575, 1.000000000000000000),
 ( 1.000000000000000000, 0.7223762446138062288, 1.000000000000000000),
 ( 1.000000000000000000, 0.7156127915551832031, 1.000000000000000000),
 ( 1.000000000000000000, 0.7133893117691495478, 1.000000000000000000),
 ( 1.000000000000000000, 0.7090389252574379464, 1.000000000000000000),
 ( 1.000000000000000000, 0.7069297463490226141, 1.000000000000000000),
 ( 1.000000000000000000, 0.7010696893203360869, 1.000000000000000000),
 ( 1.000000000000000000, 0.6977361265598307494, 1.000000000000000000),
 ( 1.000000000000000000, 0.6948030504688722520, 1.000000000000000000),
 ( 1.000000000000000000, 0.6942033558614880695, 1.000000000000000000),
 ( 1.000000000000000000, 0.6937817651809198294, 1.000000000000000000),
 ( 1.000000000000000000, 0.6939284133496614881, 1.000000000000000000),
 ( 1.000000000000000000, 0.6944177883068214374, 1.000000000000000000) ) ) 
 REPRESENTATION_ITEM ( '' )  SURFACE ( )  );
#66976=DIRECTION ( 'NONE',  ( 0.000000000000000000, -0.000000000000000000, 1.000000000000000000 ) ) ;
#66977=CARTESIAN_POINT ( 'NONE',  ( -12.09999999999999432, 12.50000000000000000, 5.088040615133786027 ) ) ;
#66978=EDGE_CURVE ( 'NONE', #91821, #83874, #61422, .T. ) ;
#66979=EDGE_CURVE ( 'NONE', #61373, #114904, #23728, .T. ) ;
#66980=CARTESIAN_POINT ( 'NONE',  ( 11.24999999999991118, 2.500000000000000000, 5.802370205355744659 ) ) ;
#66981=EDGE_CURVE ( 'NONE', #113203, #47037, #76072, .T. ) ;
#66982=ADVANCED_FACE ( 'NONE', ( #93750 ), #21801, .T. ) ;
#66983=CARTESIAN_POINT ( 'NONE',  ( -11.84999999999999787, 2.500000000000000000, -1.818653347947321919 ) ) ;
#66984=EDGE_LOOP ( 'NONE', ( #113723, #63179 ) ) ;
#66985=ORIENTED_EDGE ( 'NONE', *, *, #5145, .F. ) ;
#66986=ORIENTED_EDGE ( 'NONE', *, *, #40896, .F. ) ;
#66987=VERTEX_POINT ( 'NONE', #72825 ) ;
#66988=DIRECTION ( 'NONE',  ( 0.000000000000000000, 0.000000000000000000, 1.000000000000000000 ) ) ;
#66989=ADVANCED_FACE ( 'NONE', ( #33554 ), #113378, .T. ) ;
#66990=AXIS2_PLACEMENT_3D ( 'NONE', #37102, #126769, #68475 ) ;
#66991=DIRECTION ( 'NONE',  ( 0.000000000000000000, 1.000000000000000000, 0.000000000000000000 ) ) ;
#66992=CONICAL_SURFACE ( 'NONE', #102511, 0.1000000000000002554, 0.003490658503988666988 ) ;
#66993=EDGE_CURVE ( 'NONE', #89300, #101406, #83913, .T. ) ;
#66995=ORIENTED_EDGE ( 'NONE', *, *, #85769, .T. ) ;
#66996=VERTEX_POINT ( 'NONE', #125758 ) ;
#66997=CARTESIAN_POINT ( 'NONE',  ( -0.8000000000000381251, 2.500000000000000000, 4.330127018922196314 ) ) ;
#66998=CIRCLE ( 'NONE', #92140, 0.1000000000000002554 ) ;
#66999=ADVANCED_FACE ( 'NONE', ( #15816 ), #65570, .T. ) ;
#67000=CARTESIAN_POINT ( 'NONE',  ( 4.913542845205344456, -2.500000000001271871, 9.942462991357244206 ) ) ;
#67001=CARTESIAN_POINT ( 'NONE',  ( 4.799999999999935874, 2.500000000000000000, 0.2464101615137735679 ) ) ;
#67002=DIRECTION ( 'NONE',  ( -4.274815082592931898E-19, -0.9999939076577903929, -0.003490651415223739937 ) ) ;
#67003=CARTESIAN_POINT ( 'NONE',  ( -14.54999999999998472, 12.50000000000000000, -2.165063509461099489 ) ) ;
#67004=ADVANCED_FACE ( 'NONE', ( #55747 ), #51045, .T. ) ;
#67005=ORIENTED_EDGE ( 'NONE', *, *, #52058, .T. ) ;
#67006=ADVANCED_FACE ( 'NONE', ( #26305 ), #124189, .T. ) ;
#67007=EDGE_LOOP ( 'NONE', ( #128271, #33477, #105875, #76683 ) ) ;
#67008=EDGE_LOOP ( 'NONE', ( #119842, #57455 ) ) ;
#67009=ORIENTED_EDGE ( 'NONE', *, *, #23377, .T. ) ;
#67010=DIRECTION ( 'NONE',  ( 0.000000000000000000, 0.000000000000000000, 1.000000000000000000 ) ) ;
#67011=ORIENTED_EDGE ( 'NONE', *, *, #49356, .F. ) ;
#67012=ORIENTED_EDGE ( 'NONE', *, *, #86521, .F. ) ;
#67013=CARTESIAN_POINT ( 'NONE',  ( -0.8000000000000376810, 2.500000000000000000, -4.330127018922201643 ) ) ;
#67014=CARTESIAN_POINT ( 'NONE',  ( 11.84999999999990372, 2.500000000000000000, 1.818653347947321475 ) ) ;
#67015=FACE_OUTER_BOUND ( 'NONE', #125658, .T. ) ;
#67016=DIRECTION ( 'NONE',  ( 0.000000000000000000, 0.000000000000000000, 1.000000000000000000 ) ) ;
#67017=DIRECTION ( 'NONE',  ( 0.000000000000000000, -0.000000000000000000, 1.000000000000000000 ) ) ;
#67018=ORIENTED_EDGE ( 'NONE', *, *, #124330, .F. ) ;
#67019=DIRECTION ( 'NONE',  ( 0.000000000000000000, -0.9999939076577903929, 0.003490651415223739937 ) ) ;
#67020=CONICAL_SURFACE ( 'NONE', #81703, 0.1000000000000002554, 0.003490658503988666988 ) ;
#67021=CIRCLE ( 'NONE', #10585, 0.06509327318403745899 ) ;
#67022=VERTEX_POINT ( 'NONE', #95688 ) ;
#67023=CARTESIAN_POINT ( 'NONE',  ( -4.200000000000025935, 12.50000000000000000, 4.330127018922196314 ) ) ;
#67024=ORIENTED_EDGE ( 'NONE', *, *, #60364, .F. ) ;
#67025=CARTESIAN_POINT ( 'NONE',  ( -6.850000000000017408, 2.500000000000000000, -6.248780366869526759 ) ) ;
#67026=DIRECTION ( 'NONE',  ( -0.000000000000000000, -1.000000000000000000, -0.000000000000000000 ) ) ;
#67027=ORIENTED_EDGE ( 'NONE', *, *, #41972, .F. ) ;
#67028=CARTESIAN_POINT ( 'NONE',  ( -14.34999999999998543, 12.50000000000000000, 1.818653347947325472 ) ) ;
#67029=DIRECTION ( 'NONE',  ( 0.000000000000000000, 0.000000000000000000, -1.000000000000000000 ) ) ;
#67030=ORIENTED_EDGE ( 'NONE', *, *, #84737, .T. ) ;
#67031=EDGE_CURVE ( 'NONE', #36337, #53182, #34849, .T. ) ;
#67032=CARTESIAN_POINT ( 'NONE',  ( 14.99999999999992895, 12.50000000000000000, -0.06509327318403970719 ) ) ;
#67033=EDGE_CURVE ( 'NONE', #106863, #55645, #36122, .T. ) ;
#67034=ORIENTED_EDGE ( 'NONE', *, *, #66419, .T. ) ;
#67035=VERTEX_POINT ( 'NONE', #117222 ) ;
#67036=FACE_OUTER_BOUND ( 'NONE', #15303, .T. ) ;
#67037=DIRECTION ( 'NONE',  ( -0.000000000000000000, 1.000000000000000000, -0.000000000000000000 ) ) ;
#67040=AXIS2_PLACEMENT_3D ( 'NONE', #83047, #92866, #43771 ) ;
#67041=CONICAL_SURFACE ( 'NONE', #83787, 0.1000000000000000472, 0.003490658503988666988 ) ;
#67042=DIRECTION ( 'NONE',  ( 0.000000000000000000, 0.000000000000000000, 1.000000000000000000 ) ) ;
#67043=DIRECTION ( 'NONE',  ( 0.000000000000000000, 0.000000000000000000, -1.000000000000000000 ) ) ;
#67044=CONICAL_SURFACE ( 'NONE', #110965, 0.1000000000000002554, 0.003490658503988666988 ) ;
#67045=EDGE_LOOP ( 'NONE', ( #120999, #124649, #92860, #103220 ) ) ;
#67046=DIRECTION ( 'NONE',  ( 0.000000000000000000, 1.000000000000000000, 0.000000000000000000 ) ) ;
#67047=ORIENTED_EDGE ( 'NONE', *, *, #57367, .F. ) ;
#67048=AXIS2_PLACEMENT_3D ( 'NONE', #114778, #64397, #6731 ) ;
#67049=CARTESIAN_POINT ( 'NONE',  ( -14.34999999999998543, 12.50000000000000000, 1.818653347947325472 ) ) ;
#67050=DIRECTION ( 'NONE',  ( 0.000000000000000000, 0.000000000000000000, 1.000000000000000000 ) ) ;
#67051=DIRECTION ( 'NONE',  ( 0.000000000000000000, 1.000000000000000000, 0.000000000000000000 ) ) ;
#67052=CARTESIAN_POINT ( 'NONE',  ( 5.199999999999933564, 2.500000000000000000, 3.983716857408420076 ) ) ;
#67053=CARTESIAN_POINT ( 'NONE',  ( 3.149999999999946176, 12.50000000000000000, -2.511473670974877948 ) ) ;
#67054=VERTEX_POINT ( 'NONE', #125143 ) ;
#67055=DIRECTION ( 'NONE',  ( 0.000000000000000000, 0.000000000000000000, 1.000000000000000000 ) ) ;
#67057=ORIENTED_EDGE ( 'NONE', *, *, #94147, .T. ) ;
#67058=FACE_OUTER_BOUND ( 'NONE', #92285, .T. ) ;
#67060=ORIENTED_EDGE ( 'NONE', *, *, #65354, .F. ) ;
#67061=VERTEX_POINT ( 'NONE', #26941 ) ;
#67062=DIRECTION ( 'NONE',  ( -0.000000000000000000, -1.000000000000000000, -0.000000000000000000 ) ) ;
#67063=CIRCLE ( 'NONE', #27364, 0.06509327318403745899 ) ;
#67064=CIRCLE ( 'NONE', #69145, 0.06509327318403745899 ) ;
#67065=VERTEX_POINT ( 'NONE', #44653 ) ;
#67066=DIRECTION ( 'NONE',  ( 0.000000000000000000, 0.000000000000000000, -1.000000000000000000 ) ) ;
#67067=DIRECTION ( 'NONE',  ( 0.000000000000000000, 0.000000000000000000, -1.000000000000000000 ) ) ;
#67068=CARTESIAN_POINT ( 'NONE',  ( 1.449999999999950440, 12.50000000000000000, 6.148780366869520009 ) ) ;
#67069=ORIENTED_EDGE ( 'NONE', *, *, #64341, .T. ) ;
#67070=FACE_BOUND ( 'NONE', #76839, .T. ) ;
#67071=CARTESIAN_POINT ( 'NONE',  ( -12.04999999999999538, 2.500000000000000000, 6.595190528383296780 ) ) ;
#67072=ORIENTED_EDGE ( 'NONE', *, *, #109184, .T. ) ;
#67073=CIRCLE ( 'NONE', #113075, 0.1000000000000002554 ) ;
#67074=ADVANCED_FACE ( 'NONE', ( #17078 ), #57027, .T. ) ;
#67075=FACE_OUTER_BOUND ( 'NONE', #93232, .T. ) ;
#67076=DIRECTION ( 'NONE',  ( 0.000000000000000000, 1.000000000000000000, 0.000000000000000000 ) ) ;
#67077=EDGE_CURVE ( 'NONE', #76508, #112624, #74014, .T. ) ;
#67078=ORIENTED_EDGE ( 'NONE', *, *, #116669, .T. ) ;
#67079=ORIENTED_EDGE ( 'NONE', *, *, #118962, .F. ) ;
#67080=EDGE_LOOP ( 'NONE', ( #5161, #21669 ) ) ;
#67081=DIRECTION ( 'NONE',  ( 0.000000000000000000, 0.000000000000000000, 1.000000000000000000 ) ) ;
#67082=DIRECTION ( 'NONE',  ( -0.000000000000000000, 1.000000000000000000, -0.000000000000000000 ) ) ;
#67083=CARTESIAN_POINT ( 'NONE',  ( 3.349999999999945466, 2.500000000000000000, -2.857883832488653741 ) ) ;
#67084=EDGE_CURVE ( 'NONE', #90336, #55993, #17557, .T. ) ;
#67085=FACE_BOUND ( 'NONE', #107049, .T. ) ;
#67086=EDGE_LOOP ( 'NONE', ( #120876, #16349 ) ) ;
#67087=CARTESIAN_POINT ( 'NONE',  ( 4.399999999999940847, 2.500000000000000000, -4.083716857408426826 ) ) ;
#67088=DIRECTION ( 'NONE',  ( 0.000000000000000000, 1.000000000000000000, 0.000000000000000000 ) ) ;
#67089=EDGE_LOOP ( 'NONE', ( #68974, #64991, #13936, #42912 ) ) ;
#67090=CONICAL_SURFACE ( 'NONE', #33683, 0.1000000000000000472, 0.003490658503988666988 ) ;
#67091=CARTESIAN_POINT ( 'NONE',  ( -8.350000000000013856, 2.500000000000000000, -2.265063509461101798 ) ) ;
#67092=DIRECTION ( 'NONE',  ( -0.000000000000000000, 1.000000000000000000, -0.000000000000000000 ) ) ;
#67093=DIRECTION ( 'NONE',  ( 0.000000000000000000, 1.000000000000000000, 0.000000000000000000 ) ) ;
#67094=DIRECTION ( 'NONE',  ( 0.000000000000000000, 1.000000000000000000, 0.000000000000000000 ) ) ;
#67095=FACE_OUTER_BOUND ( 'NONE', #90245, .T. ) ;
#67096=CIRCLE ( 'NONE', #100571, 0.06509327318403745899 ) ;
#67097=CIRCLE ( 'NONE', #96362, 0.06509327318403745899 ) ;
#67098=ORIENTED_EDGE ( 'NONE', *, *, #112359, .F. ) ;
#67099=EDGE_LOOP ( 'NONE', ( #18066, #55102, #80325, #125689 ) ) ;
#67100=ORIENTED_EDGE ( 'NONE', *, *, #38919, .F. ) ;
#67101=ORIENTED_EDGE ( 'NONE', *, *, #21276, .T. ) ;
#67102=ORIENTED_EDGE ( 'NONE', *, *, #52052, .F. ) ;
#67103=DIRECTION ( 'NONE',  ( 0.000000000000000000, -0.000000000000000000, 1.000000000000000000 ) ) ;
#67104=DIRECTION ( 'NONE',  ( -0.000000000000000000, 1.000000000000000000, -0.000000000000000000 ) ) ;
#67105=ORIENTED_EDGE ( 'NONE', *, *, #26222, .F. ) ;
#67106=FACE_BOUND ( 'NONE', #64201, .T. ) ;
#67107=CARTESIAN_POINT ( 'NONE',  ( 13.09999999999990195, 2.500000000000000000, -4.676537180435978769 ) ) ;
#67108=AXIS2_PLACEMENT_3D ( 'NONE', #28250, #19726, #30202 ) ;
#67109=EDGE_CURVE ( 'NONE', #36921, #103404, #111570, .T. ) ;
#67110=DIRECTION ( 'NONE',  ( 0.000000000000000000, -0.9999939076577903929, 0.003490651415223739937 ) ) ;
#67111=PLANE ( 'NONE',  #64123 ) ;
#67112=DIRECTION ( 'NONE',  ( 0.000000000000000000, -0.000000000000000000, 1.000000000000000000 ) ) ;
#67113=EDGE_CURVE ( 'NONE', #90160, #63978, #38436, .T. ) ;
#67114=LINE ( 'NONE', #46878, #22482 ) ;
#67115=ORIENTED_EDGE ( 'NONE', *, *, #53674, .F. ) ;
#67116=CARTESIAN_POINT ( 'NONE',  ( 9.999999999999911182, 12.50000000000000000, -3.637306695894650055 ) ) ;
#67117=EDGE_CURVE ( 'NONE', #53996, #43807, #109525, .T. ) ;
#67118=AXIS2_PLACEMENT_3D ( 'NONE', #27974, #40389, #77703 ) ;
#67119=VERTEX_POINT ( 'NONE', #77325 ) ;
#67120=AXIS2_PLACEMENT_3D ( 'NONE', #110893, #2223, #40237 ) ;
#67121=ORIENTED_EDGE ( 'NONE', *, *, #107948, .T. ) ;
#67122=ORIENTED_EDGE ( 'NONE', *, *, #33726, .F. ) ;
#67123=EDGE_CURVE ( 'NONE', #102800, #60587, #71879, .T. ) ;
#67124=CARTESIAN_POINT ( 'NONE',  ( 5.849999999999935696, 12.50000000000000000, -7.188010851410854052 ) ) ;
#67126=EDGE_CURVE ( 'NONE', #48660, #98142, #119989, .T. ) ;
#67127=DIRECTION ( 'NONE',  ( 0.000000000000000000, 0.000000000000000000, 1.000000000000000000 ) ) ;
#67128=EDGE_CURVE ( 'NONE', #120619, #79607, #2915, .T. ) ;
#67129=EDGE_LOOP ( 'NONE', ( #38258, #104743 ) ) ;
#67130=CARTESIAN_POINT ( 'NONE',  ( 11.24999999999994316, 2.500000000000000000, -6.595190528383302109 ) ) ;
#67131=CIRCLE ( 'NONE', #60901, 0.09999999999999982514 ) ;
#67132=EDGE_CURVE ( 'NONE', #57691, #73360, #44776, .T. ) ;
#67133=DIRECTION ( 'NONE',  ( -0.000000000000000000, 1.000000000000000000, -0.000000000000000000 ) ) ;
#67134=DIRECTION ( 'NONE',  ( -0.000000000000000000, -1.000000000000000000, -0.000000000000000000 ) ) ;
#67135=EDGE_CURVE ( 'NONE', #80417, #34203, #117914, .T. ) ;
#67136=AXIS2_PLACEMENT_3D ( 'NONE', #118003, #127828, #57809 ) ;
#67137=AXIS2_PLACEMENT_3D ( 'NONE', #122912, #5689, #45644 ) ;
#67139=DIRECTION ( 'NONE',  ( 0.000000000000000000, 0.000000000000000000, 1.000000000000000000 ) ) ;
#67140=PLANE ( 'NONE',  #86378 ) ;
#67141=CARTESIAN_POINT ( 'NONE',  ( -6.900000000000019007, 12.50000000000000000, -4.048810130592463530 ) ) ;
#67142=ORIENTED_EDGE ( 'NONE', *, *, #121284, .F. ) ;
#67143=CARTESIAN_POINT ( 'NONE',  ( 1.249999999999952038, 2.500000000000000000, -1.572243186433550211 ) ) ;
#67144=ADVANCED_FACE ( 'NONE', ( #115821 ), #34320, .T. ) ;
#67145=EDGE_LOOP ( 'NONE', ( #95365, #46333 ) ) ;
#67146=ORIENTED_EDGE ( 'NONE', *, *, #33067, .F. ) ;
#67147=CARTESIAN_POINT ( 'NONE',  ( -6.700000000000016165, 2.500000000000000000, 4.330127018922196314 ) ) ;
#67148=CARTESIAN_POINT ( 'NONE',  ( -2.050000000000032685, 2.500000000000000000, -6.495190528383302464 ) ) ;
#67149=CARTESIAN_POINT ( 'NONE',  ( 10.39999999999991154, 2.500000000000000000, -5.022947341949754119 ) ) ;
#67150=VERTEX_POINT ( 'NONE', #75254 ) ;
#67151=ORIENTED_EDGE ( 'NONE', *, *, #124899, .T. ) ;
#67152=CARTESIAN_POINT ( 'NONE',  ( 11.24999999999994316, 12.50000000000000000, 2.230156782645134950 ) ) ;
#67153=DIRECTION ( 'NONE',  ( -0.000000000000000000, 1.000000000000000000, -0.000000000000000000 ) ) ;
#67154=CARTESIAN_POINT ( 'NONE',  ( 16.56576425165007649, -1.499999999999997113, -6.084390597445789695 ) ) ;
#67155=ORIENTED_EDGE ( 'NONE', *, *, #15919, .T. ) ;
#67156=ORIENTED_EDGE ( 'NONE', *, *, #47704, .F. ) ;
#67157=VECTOR ( 'NONE', #38082, 1000.000000000000000 ) ;
#67158=CIRCLE ( 'NONE', #12794, 0.06509327318403745899 ) ;
#67159=CARTESIAN_POINT ( 'NONE',  ( -14.34999999999998543, 2.500000000000000000, 1.818653347947325472 ) ) ;
#67160=ORIENTED_EDGE ( 'NONE', *, *, #94771, .F. ) ;
#67161=CARTESIAN_POINT ( 'NONE',  ( 0.8499999999999553468, 2.500000000000000000, -2.265063509461101798 ) ) ;
#67162=CIRCLE ( 'NONE', #8591, 0.1000000000000002554 ) ;
#67163=FACE_OUTER_BOUND ( 'NONE', #27087, .T. ) ;
#67164=ORIENTED_EDGE ( 'NONE', *, *, #121380, .T. ) ;
#67165=CARTESIAN_POINT ( 'NONE',  ( -0.6500000000000389910, 2.500000000000000000, -1.918653347947326004 ) ) ;
#67166=AXIS2_PLACEMENT_3D ( 'NONE', #126750, #77626, #97918 ) ;
#67167=PLANE ( 'NONE',  #58856 ) ;
#67168=DIRECTION ( 'NONE',  ( 0.000000000000000000, 0.000000000000000000, 1.000000000000000000 ) ) ;
#67169=CIRCLE ( 'NONE', #92230, 0.09999999999999982514 ) ;
#67170=DIRECTION ( 'NONE',  ( -0.000000000000000000, -1.000000000000000000, -0.000000000000000000 ) ) ;
#67171=ORIENTED_EDGE ( 'NONE', *, *, #119965, .T. ) ;
#67172=DIRECTION ( 'NONE',  ( -0.000000000000000000, 1.000000000000000000, -0.000000000000000000 ) ) ;
#67173=ADVANCED_FACE ( 'NONE', ( #83782 ), #32179, .T. ) ;
#67174=DIRECTION ( 'NONE',  ( 0.000000000000000000, 0.000000000000000000, 1.000000000000000000 ) ) ;
#67175=VERTEX_POINT ( 'NONE', #105363 ) ;
#67176=EDGE_LOOP ( 'NONE', ( #63287, #8431 ) ) ;
#67178=DIRECTION ( 'NONE',  ( 0.000000000000000000, 0.000000000000000000, -1.000000000000000000 ) ) ;
#67179=DIRECTION ( 'NONE',  ( 0.000000000000000000, 0.000000000000000000, 1.000000000000000000 ) ) ;
#67180=FACE_OUTER_BOUND ( 'NONE', #38198, .T. ) ;
#67181=DIRECTION ( 'NONE',  ( -0.000000000000000000, 1.000000000000000000, -0.000000000000000000 ) ) ;
#67182=DIRECTION ( 'NONE',  ( 0.000000000000000000, 1.000000000000000000, 0.000000000000000000 ) ) ;
#67183=EDGE_CURVE ( 'NONE', #5504, #106259, #65599, .T. ) ;
#67184=CARTESIAN_POINT ( 'NONE',  ( 16.98389417446983884, 2.499999999999060751, -5.627887362476348798 ) ) ;
#67185=CARTESIAN_POINT ( 'NONE',  ( 11.04999999999990834, 12.50000000000000000, 1.883746621131358934 ) ) ;
#67186=DIRECTION ( 'NONE',  ( 0.000000000000000000, 0.000000000000000000, 1.000000000000000000 ) ) ;
#67187=DIRECTION ( 'NONE',  ( 0.000000000000000000, -0.9999939076577903929, 0.003490651415223739937 ) ) ;
#67188=AXIS2_PLACEMENT_3D ( 'NONE', #64016, #33911, #64655 ) ;
#67189=AXIS2_PLACEMENT_3D ( 'NONE', #99096, #38245, #118722 ) ;
#67190=ORIENTED_EDGE ( 'NONE', *, *, #29692, .T. ) ;
#67191=DIRECTION ( 'NONE',  ( 0.000000000000000000, 0.000000000000000000, 1.000000000000000000 ) ) ;
#67192=CARTESIAN_POINT ( 'NONE',  ( 4.149999999999939959, 12.50000000000000000, 2.922977105672686982 ) ) ;
#67193=DIRECTION ( 'NONE',  ( 0.000000000000000000, 0.000000000000000000, 1.000000000000000000 ) ) ;
#67194=CARTESIAN_POINT ( 'NONE',  ( 4.349999999999940137, 12.50000000000000000, -6.906693963081115939 ) ) ;
#67195=AXIS2_PLACEMENT_3D ( 'NONE', #60198, #18944, #20899 ) ;
#67196=CIRCLE ( 'NONE', #71332, 0.1000000000000002554 ) ;
#67197=ORIENTED_EDGE ( 'NONE', *, *, #75599, .T. ) ;
#67198=DIRECTION ( 'NONE',  ( 0.000000000000000000, 0.000000000000000000, 1.000000000000000000 ) ) ;
#67199=CONICAL_SURFACE ( 'NONE', #63040, 0.1000000000000002554, 0.003490658503988666988 ) ;
#67200=DIRECTION ( 'NONE',  ( 0.000000000000000000, 0.000000000000000000, 1.000000000000000000 ) ) ;
#67201=CARTESIAN_POINT ( 'NONE',  ( -0.8000000000000376810, 12.50000000000000000, -4.330127018922201643 ) ) ;
#67203=CIRCLE ( 'NONE', #27514, 0.06509327318403745899 ) ;
#67204=ORIENTED_EDGE ( 'NONE', *, *, #88134, .T. ) ;
#67205=CONICAL_SURFACE ( 'NONE', #14984, 0.1000000000000002554, 0.003490658503988666988 ) ;
#67206=EDGE_CURVE ( 'NONE', #126098, #78919, #113904, .T. ) ;
#67207=ORIENTED_EDGE ( 'NONE', *, *, #40464, .T. ) ;
#67208=ORIENTED_EDGE ( 'NONE', *, *, #84766, .F. ) ;
#67209=AXIS2_PLACEMENT_3D ( 'NONE', #107812, #108446, #79636 ) ;
#67210=EDGE_LOOP ( 'NONE', ( #54389, #64754 ) ) ;
#67211=CARTESIAN_POINT ( 'NONE',  ( 9.999999999999912959, 2.500000000000000000, -5.022947341949754119 ) ) ;
#67212=VECTOR ( 'NONE', #42848, 1000.000000000000000 ) ;
#67213=DIRECTION ( 'NONE',  ( 0.000000000000000000, -0.000000000000000000, 1.000000000000000000 ) ) ;
#67214=CARTESIAN_POINT ( 'NONE',  ( 6.849999999999929479, 2.500000000000000000, -1.718653347947326049 ) ) ;
#67215=CARTESIAN_POINT ( 'NONE',  ( 8.349999999999923261, 12.50000000000000000, 2.857883832488649301 ) ) ;
#67216=EDGE_CURVE ( 'NONE', #127598, #119087, #7087, .T. ) ;
#67217=ORIENTED_EDGE ( 'NONE', *, *, #104684, .T. ) ;
#67218=CIRCLE ( 'NONE', #40078, 0.09999999999999982514 ) ;
#67219=CARTESIAN_POINT ( 'NONE',  ( -2.500000000000030642, 2.500000000000000000, -5.122947341949753763 ) ) ;
#67220=EDGE_LOOP ( 'NONE', ( #49643, #119271 ) ) ;
#67221=CARTESIAN_POINT ( 'NONE',  ( 48.67919755221870304, -3.179368040587171151, -5.083101271994035386 ) ) ;
#67222=CARTESIAN_POINT ( 'NONE',  ( 16.56576425165006228, -1.499999999999999778, -6.084390597445814564 ) ) ;
#67223=EDGE_CURVE ( 'NONE', #59349, #23039, #115767, .T. ) ;
#67224=CARTESIAN_POINT ( 'NONE',  ( 5.649999999999934630, 12.50000000000000000, 6.148780366869520897 ) ) ;
#67225=DIRECTION ( 'NONE',  ( 0.000000000000000000, 1.000000000000000000, 0.000000000000000000 ) ) ;
#67226=EDGE_CURVE ( 'NONE', #55758, #79598, #123687, .T. ) ;
#67227=EDGE_LOOP ( 'NONE', ( #3908, #102355, #129371, #96674 ) ) ;
#67228=ORIENTED_EDGE ( 'NONE', *, *, #60524, .T. ) ;
#67229=EDGE_CURVE ( 'NONE', #30373, #62733, #59370, .T. ) ;
#67230=ORIENTED_EDGE ( 'NONE', *, *, #51387, .T. ) ;
#67231=ORIENTED_EDGE ( 'NONE', *, *, #45501, .T. ) ;
#67232=LINE ( 'NONE', #58748, #98443 ) ;
#67233=DIRECTION ( 'NONE',  ( -0.000000000000000000, 1.000000000000000000, -0.000000000000000000 ) ) ;
#67234=DIRECTION ( 'NONE',  ( 0.000000000000000000, 0.000000000000000000, -1.000000000000000000 ) ) ;
#67235=EDGE_CURVE ( 'NONE', #117751, #102540, #126296, .T. ) ;
#67236=FACE_BOUND ( 'NONE', #31764, .T. ) ;
#67237=DIRECTION ( 'NONE',  ( 0.000000000000000000, -0.9999939076577903929, 0.003490651415223739937 ) ) ;
#67238=CARTESIAN_POINT ( 'NONE',  ( 10.19999999999991402, 12.50000000000000000, 0.3464101615137735735 ) ) ;
#67239=CARTESIAN_POINT ( 'NONE',  ( 3.149999999999946176, 12.50000000000000000, -6.841600689897077814 ) ) ;
#67240=PLANE ( 'NONE',  #20771 ) ;
#67241=AXIS2_PLACEMENT_3D ( 'NONE', #51678, #102060, #71292 ) ;
#67242=AXIS2_PLACEMENT_3D ( 'NONE', #5710, #126797, #115016 ) ;
#67244=AXIS2_PLACEMENT_3D ( 'NONE', #15180, #123857, #35506 ) ;
#67245=DIRECTION ( 'NONE',  ( 0.000000000000000000, 0.000000000000000000, -1.000000000000000000 ) ) ;
#67246=CARTESIAN_POINT ( 'NONE',  ( 87.50000000000001421, 0.000000000000000000, 0.000000000000000000 ) ) ;
#67247=DIRECTION ( 'NONE',  ( 0.000000000000000000, 0.000000000000000000, 1.000000000000000000 ) ) ;
#67248=ORIENTED_EDGE ( 'NONE', *, *, #80343, .F. ) ;
#67249=VERTEX_POINT ( 'NONE', #24870 ) ;
#67250=VERTEX_POINT ( 'NONE', #115146 ) ;
#67251=EDGE_LOOP ( 'NONE', ( #39700, #29215 ) ) ;
#67252=AXIS2_PLACEMENT_3D ( 'NONE', #126069, #36435, #76345 ) ;
#67253=VECTOR ( 'NONE', #13957, 1000.000000000000000 ) ;
#67254=DIRECTION ( 'NONE',  ( 0.000000000000000000, 0.000000000000000000, 1.000000000000000000 ) ) ;
#67255=FACE_BOUND ( 'NONE', #17605, .T. ) ;
#67256=LINE ( 'NONE', #97398, #89172 ) ;
#67258=ORIENTED_EDGE ( 'NONE', *, *, #113394, .T. ) ;
#67259=DIRECTION ( 'NONE',  ( -4.274815082592931898E-19, -0.9999939076577903929, -0.003490651415223739937 ) ) ;
#67260=FACE_OUTER_BOUND ( 'NONE', #60688, .T. ) ;
#67261=DIRECTION ( 'NONE',  ( -0.000000000000000000, -1.000000000000000000, -0.000000000000000000 ) ) ;
#67262=VERTEX_POINT ( 'NONE', #34714 ) ;
#67263=CARTESIAN_POINT ( 'NONE',  ( 3.949999999999939782, 2.500000000000000000, 2.411473670974873862 ) ) ;
#67264=CARTESIAN_POINT ( 'NONE',  ( -9.150000000000009237, 12.50000000000000000, -6.495190528383297135 ) ) ;
#67265=EDGE_CURVE ( 'NONE', #49835, #76293, #106011, .T. ) ;
#67266=ADVANCED_FACE ( 'NONE', ( #5852 ), #86525, .T. ) ;
#67267=ORIENTED_EDGE ( 'NONE', *, *, #34854, .F. ) ;
#67268=EDGE_CURVE ( 'NONE', #2954, #34969, #13360, .T. ) ;
#67269=DIRECTION ( 'NONE',  ( 0.000000000000000000, 0.000000000000000000, 1.000000000000000000 ) ) ;
#67270=LINE ( 'NONE', #39173, #112477 ) ;
#67271=EDGE_CURVE ( 'NONE', #97516, #98415, #43884, .T. ) ;
#67272=ADVANCED_FACE ( 'NONE', ( #45165 ), #104076, .T. ) ;
#67274=AXIS2_PLACEMENT_3D ( 'NONE', #71552, #111476, #21832 ) ;
#67275=ORIENTED_EDGE ( 'NONE', *, *, #110626, .T. ) ;
#67276=CARTESIAN_POINT ( 'NONE',  ( 0.5999999999999551248, 12.50000000000000000, -4.676537180435978769 ) ) ;
#67277=DIRECTION ( 'NONE',  ( 0.000000000000000000, 1.000000000000000000, 0.000000000000000000 ) ) ;
#67278=VERTEX_POINT ( 'NONE', #54329 ) ;
#67279=DIRECTION ( 'NONE',  ( 0.000000000000000000, 0.000000000000000000, 1.000000000000000000 ) ) ;
#67280=EDGE_CURVE ( 'NONE', #113021, #127796, #74114, .T. ) ;
#67281=ORIENTED_EDGE ( 'NONE', *, *, #19568, .F. ) ;
#67282=VERTEX_POINT ( 'NONE', #4544 ) ;
#67283=CARTESIAN_POINT ( 'NONE',  ( -8.300000000000009592, 12.50000000000000000, 4.265033745738159077 ) ) ;
#67284=CIRCLE ( 'NONE', #107013, 0.06509327318403745899 ) ;
#67285=ORIENTED_EDGE ( 'NONE', *, *, #26923, .F. ) ;
#67286=DIRECTION ( 'NONE',  ( 0.000000000000000000, 0.000000000000000000, 1.000000000000000000 ) ) ;
#67287=AXIS2_PLACEMENT_3D ( 'NONE', #3604, #86003, #4229 ) ;
#67288=FACE_BOUND ( 'NONE', #20400, .T. ) ;
#67289=ADVANCED_FACE ( 'NONE', ( #125630 ), #75895, .T. ) ;
#67290=CIRCLE ( 'NONE', #98704, 0.1000000000000002554 ) ;
#67291=EDGE_CURVE ( 'NONE', #68087, #120638, #71972, .T. ) ;
#67292=ORIENTED_EDGE ( 'NONE', *, *, #89902, .F. ) ;
#67293=AXIS2_PLACEMENT_3D ( 'NONE', #43592, #83511, #123410 ) ;
#67294=CARTESIAN_POINT ( 'NONE',  ( 8.749999999999918288, 2.500000000000000000, -1.372243186433550033 ) ) ;
#67296=CARTESIAN_POINT ( 'NONE',  ( 2.099999999999950351, 12.50000000000000000, -5.022947341949754119 ) ) ;
#67298=LINE ( 'NONE', #107256, #44543 ) ;
#67299=DIRECTION ( 'NONE',  ( -0.000000000000000000, -1.000000000000000000, -0.000000000000000000 ) ) ;
#67300=DIRECTION ( 'NONE',  ( -0.000000000000000000, -1.000000000000000000, -0.000000000000000000 ) ) ;
#67301=CIRCLE ( 'NONE', #100766, 0.09999999999999982514 ) ;
#67302=VERTEX_POINT ( 'NONE', #58216 ) ;
#67303=ORIENTED_EDGE ( 'NONE', *, *, #18080, .T. ) ;
#67304=PLANE ( 'NONE',  #55906 ) ;
#67305=DIRECTION ( 'NONE',  ( -0.000000000000000000, 1.000000000000000000, -0.000000000000000000 ) ) ;
#67306=CIRCLE ( 'NONE', #125818, 0.06509327318403745899 ) ;
#67307=AXIS2_PLACEMENT_3D ( 'NONE', #4081, #73463, #104222 ) ;
#67308=AXIS2_PLACEMENT_3D ( 'NONE', #38030, #10491, #127696 ) ;
#67309=DIRECTION ( 'NONE',  ( -0.000000000000000000, 1.000000000000000000, -0.000000000000000000 ) ) ;
#67310=ORIENTED_EDGE ( 'NONE', *, *, #116811, .F. ) ;
#67311=ORIENTED_EDGE ( 'NONE', *, *, #30723, .T. ) ;
#67312=ORIENTED_EDGE ( 'NONE', *, *, #59381, .T. ) ;
#67313=DIRECTION ( 'NONE',  ( 0.000000000000000000, 0.000000000000000000, 1.000000000000000000 ) ) ;
#67314=CIRCLE ( 'NONE', #61093, 0.06509327318403745899 ) ;
#67315=FACE_OUTER_BOUND ( 'NONE', #25546, .T. ) ;
#67316=PLANE ( 'NONE',  #95887 ) ;
#67318=CARTESIAN_POINT ( 'NONE',  ( -4.550000000000022915, 2.500000000000000000, -2.065063509461102065 ) ) ;
#67319=AXIS2_PLACEMENT_3D ( 'NONE', #121230, #2086, #42033 ) ;
#67320=CARTESIAN_POINT ( 'NONE',  ( 13.14999999999989733, 12.50000000000000000, -2.576566944158915184 ) ) ;
#67321=CARTESIAN_POINT ( 'NONE',  ( 5.599999999999934808, 2.500000000000000000, -4.083716857408426826 ) ) ;
#67322=FACE_OUTER_BOUND ( 'NONE', #125642, .T. ) ;
#67323=CARTESIAN_POINT ( 'NONE',  ( -4.550000000000022915, 2.500000000000000000, 6.595190528383296780 ) ) ;
#67324=CARTESIAN_POINT ( 'NONE',  ( 0.3999999999999563904, 12.50000000000000000, 3.637306695894644726 ) ) ;
#67325=VERTEX_POINT ( 'NONE', #129544 ) ;
#67326=ORIENTED_EDGE ( 'NONE', *, *, #59904, .T. ) ;
#67327=FACE_OUTER_BOUND ( 'NONE', #41276, .T. ) ;
#67328=VERTEX_POINT ( 'NONE', #98750 ) ;
#67329=EDGE_LOOP ( 'NONE', ( #23946, #121878, #54788, #117911 ) ) ;
#67330=DIRECTION ( 'NONE',  ( -0.000000000000000000, 1.000000000000000000, -0.000000000000000000 ) ) ;
#67331=CARTESIAN_POINT ( 'NONE',  ( -11.25000000000000178, 12.50000000000000000, -5.867463478539783672 ) ) ;
#67332=CARTESIAN_POINT ( 'NONE',  ( 11.84999999999990727, 12.50000000000000000, -1.818653347947326138 ) ) ;
#67333=PLANE ( 'NONE',  #17016 ) ;
#67334=EDGE_CURVE ( 'NONE', #111831, #3112, #90824, .T. ) ;
#67335=LINE ( 'NONE', #107293, #19333 ) ;
#67336=CARTESIAN_POINT ( 'NONE',  ( -1.700000000000035261, 2.500000000000000000, 4.230127018922196669 ) ) ;
#67337=AXIS2_PLACEMENT_3D ( 'NONE', #22711, #102535, #12845 ) ;
#67338=CARTESIAN_POINT ( 'NONE',  ( 3.749999999999975131, 2.500000000000000000, 6.395190528383296602 ) ) ;
#67339=VERTEX_POINT ( 'NONE', #88949 ) ;
#67340=PLANE ( 'NONE',  #43571 ) ;
#67342=VECTOR ( 'NONE', #49840, 1000.000000000000000 ) ;
#67343=CARTESIAN_POINT ( 'NONE',  ( 1.899999999999951283, 12.50000000000000000, 0.3464101615137736845 ) ) ;
#67344=AXIS2_PLACEMENT_3D ( 'NONE', #115054, #45067, #5110 ) ;
#67345=VERTEX_POINT ( 'NONE', #67331 ) ;
#67346=CIRCLE ( 'NONE', #75977, 0.06509327318403745899 ) ;
#67347=AXIS2_PLACEMENT_3D ( 'NONE', #8561, #48511, #50438 ) ;
#67348=ORIENTED_EDGE ( 'NONE', *, *, #59850, .F. ) ;
#67349=CIRCLE ( 'NONE', #58987, 0.1000000000000002554 ) ;
#67350=AXIS2_PLACEMENT_3D ( 'NONE', #66055, #47082, #4530 ) ;
#67351=EDGE_LOOP ( 'NONE', ( #60372, #35452, #61483, #66355 ) ) ;
#67352=ORIENTED_EDGE ( 'NONE', *, *, #78463, .T. ) ;
#67353=DIRECTION ( 'NONE',  ( 0.000000000000000000, -0.000000000000000000, 1.000000000000000000 ) ) ;
#67354=DIRECTION ( 'NONE',  ( 0.000000000000000000, -0.000000000000000000, 1.000000000000000000 ) ) ;
#67355=AXIS2_PLACEMENT_3D ( 'NONE', #13592, #82370, #103288 ) ;
#67356=ORIENTED_EDGE ( 'NONE', *, *, #85429, .F. ) ;
#67357=FACE_OUTER_BOUND ( 'NONE', #31003, .T. ) ;
#67358=DIRECTION ( 'NONE',  ( 0.000000000000000000, 0.000000000000000000, 1.000000000000000000 ) ) ;
#67359=DIRECTION ( 'NONE',  ( -0.000000000000000000, -1.000000000000000000, -0.000000000000000000 ) ) ;
#67360=ORIENTED_EDGE ( 'NONE', *, *, #16686, .T. ) ;
#67361=PLANE ( 'NONE',  #128948 ) ;
#67362=PLANE ( 'NONE',  #31190 ) ;
#67363=EDGE_LOOP ( 'NONE', ( #50015, #85594, #114656, #44344 ) ) ;
#67364=ORIENTED_EDGE ( 'NONE', *, *, #128566, .F. ) ;
#67365=EDGE_LOOP ( 'NONE', ( #72235, #88901 ) ) ;
#67366=DIRECTION ( 'NONE',  ( 0.000000000000000000, 0.000000000000000000, 1.000000000000000000 ) ) ;
#67367=AXIS2_PLACEMENT_3D ( 'NONE', #90579, #78858, #99771 ) ;
#67368=CARTESIAN_POINT ( 'NONE',  ( 8.949999999999921130, 2.500000000000000000, -6.941600689897078347 ) ) ;
#67369=EDGE_CURVE ( 'NONE', #77424, #89750, #113817, .T. ) ;
#67370=EDGE_LOOP ( 'NONE', ( #35435, #51609 ) ) ;
#67371=CARTESIAN_POINT ( 'NONE',  ( 3.549999999999940314, 12.50000000000000000, 6.841600689897072485 ) ) ;
#67373=EDGE_CURVE ( 'NONE', #50205, #61413, #99153, .T. ) ;
#67374=DIRECTION ( 'NONE',  ( -0.000000000000000000, 1.000000000000000000, -0.000000000000000000 ) ) ;
#67376=VECTOR ( 'NONE', #23969, 1000.000000000000000 ) ;
#67377=EDGE_CURVE ( 'NONE', #1255, #76788, #57381, .T. ) ;
#67378=AXIS2_PLACEMENT_3D ( 'NONE', #61085, #41469, #80080 ) ;
#67379=VERTEX_POINT ( 'NONE', #39236 ) ;
#67380=DIRECTION ( 'NONE',  ( -0.000000000000000000, -1.000000000000000000, -0.000000000000000000 ) ) ;
#67381=CONICAL_SURFACE ( 'NONE', #42392, 0.09999999999999999167, 0.003490658503988666988 ) ;
#67382=ORIENTED_EDGE ( 'NONE', *, *, #98076, .F. ) ;
#67383=EDGE_CURVE ( 'NONE', #11772, #80189, #25996, .T. ) ;
#67384=ADVANCED_FACE ( 'NONE', ( #29395 ), #7185, .T. ) ;
#67385=ORIENTED_EDGE ( 'NONE', *, *, #12454, .T. ) ;
#67386=DIRECTION ( 'NONE',  ( 0.000000000000000000, 0.000000000000000000, 1.000000000000000000 ) ) ;
#67387=EDGE_CURVE ( 'NONE', #97216, #129104, #67837, .T. ) ;
#67388=DIRECTION ( 'NONE',  ( 0.000000000000000000, 0.000000000000000000, 1.000000000000000000 ) ) ;
#67389=EDGE_CURVE ( 'NONE', #127947, #31361, #39869, .T. ) ;
#67390=EDGE_CURVE ( 'NONE', #121812, #113368, #96818, .T. ) ;
#67391=FACE_BOUND ( 'NONE', #126169, .T. ) ;
#67392=LINE ( 'NONE', #117146, #101521 ) ;
#67393=AXIS2_PLACEMENT_3D ( 'NONE', #20265, #9800, #58907 ) ;
#67394=CARTESIAN_POINT ( 'NONE',  ( -6.050000000000020250, 2.500000000000000000, -2.411473670974877859 ) ) ;
#67395=CONICAL_SURFACE ( 'NONE', #10973, 0.1000000000000002554, 0.003490658503988666988 ) ;
#67396=DIRECTION ( 'NONE',  ( -0.000000000000000000, 1.000000000000000000, -0.000000000000000000 ) ) ;
#67397=CIRCLE ( 'NONE', #521, 0.09999999999999982514 ) ;
#67398=VECTOR ( 'NONE', #22312, 1000.000000000000000 ) ;
#67399=AXIS2_PLACEMENT_3D ( 'NONE', #20967, #1958, #41912 ) ;
#67400=ORIENTED_EDGE ( 'NONE', *, *, #81365, .T. ) ;
#67401=CARTESIAN_POINT ( 'NONE',  ( -8.750000000000008882, 2.500000000000000000, -2.757883832488654097 ) ) ;
#67402=DIRECTION ( 'NONE',  ( 0.000000000000000000, 0.000000000000000000, 1.000000000000000000 ) ) ;
#67403=EDGE_CURVE ( 'NONE', #107678, #120135, #65684, .T. ) ;
#67404=CARTESIAN_POINT ( 'NONE',  ( 14.34999999999989306, 2.500000000000000000, -2.511473670974877948 ) ) ;
#67405=CIRCLE ( 'NONE', #25670, 0.1000000000000002554 ) ;
#67406=CARTESIAN_POINT ( 'NONE',  ( -3.950000000000026379, 2.500000000000000000, 2.411473670974873862 ) ) ;
#67407=EDGE_LOOP ( 'NONE', ( #12990, #33191, #47753, #44122 ) ) ;
#67408=CARTESIAN_POINT ( 'NONE',  ( 3.349999999999944578, 12.50000000000000000, -5.737276932171712751 ) ) ;
#67410=AXIS2_PLACEMENT_3D ( 'NONE', #11762, #12404, #121079 ) ;
#67411=VERTEX_POINT ( 'NONE', #117093 ) ;
#67412=DIRECTION ( 'NONE',  ( -0.000000000000000000, 1.000000000000000000, -0.000000000000000000 ) ) ;
#67413=CARTESIAN_POINT ( 'NONE',  ( -12.09999999999999609, 2.500000000000000000, -0.7928203230275502333 ) ) ;
#67414=FACE_BOUND ( 'NONE', #100850, .T. ) ;
#67415=DIRECTION ( 'NONE',  ( 0.000000000000000000, 0.000000000000000000, 1.000000000000000000 ) ) ;
#67416=ORIENTED_EDGE ( 'NONE', *, *, #128664, .F. ) ;
#67417=PLANE ( 'NONE',  #46590 ) ;
#67418=VERTEX_POINT ( 'NONE', #66711 ) ;
#67419=VERTEX_POINT ( 'NONE', #7141 ) ;
#67420=CARTESIAN_POINT ( 'NONE',  ( 19.52519901027835658, 0.5909487300084670380, -4.333354523369935762 ) ) ;
#67421=CIRCLE ( 'NONE', #23631, 0.06509327318403741736 ) ;
#67423=ORIENTED_EDGE ( 'NONE', *, *, #38207, .T. ) ;
#67424=CARTESIAN_POINT ( 'NONE',  ( -8.150000000000009237, 2.500000000000000000, 6.148780366869520009 ) ) ;
#67425=LINE ( 'NONE', #68748, #17695 ) ;
#67426=AXIS2_PLACEMENT_3D ( 'NONE', #44770, #2235, #24474 ) ;
#67427=AXIS2_PLACEMENT_3D ( 'NONE', #1044, #81545, #113586 ) ;
#67428=EDGE_CURVE ( 'NONE', #123090, #42074, #943, .T. ) ;
#67430=EDGE_CURVE ( 'NONE', #39604, #116494, #115862, .T. ) ;
#67431=AXIS2_PLACEMENT_3D ( 'NONE', #33420, #123076, #85075 ) ;
#67432=CONICAL_SURFACE ( 'NONE', #105019, 0.09999999999999982514, 0.003490658503988666988 ) ;
#67433=VERTEX_POINT ( 'NONE', #78504 ) ;
#67434=EDGE_CURVE ( 'NONE', #122576, #67250, #47740, .T. ) ;
#67435=AXIS2_PLACEMENT_3D ( 'NONE', #35684, #106349, #16656 ) ;
#67437=DIRECTION ( 'NONE',  ( 0.000000000000000000, 1.000000000000000000, 0.000000000000000000 ) ) ;
#67438=DIRECTION ( 'NONE',  ( 0.000000000000000000, 1.000000000000000000, 0.000000000000000000 ) ) ;
#67439=VECTOR ( 'NONE', #53187, 1000.000000000000000 ) ;
#67440=CARTESIAN_POINT ( 'NONE',  ( 12.04999999999990479, 2.500000000000000000, -6.495190528383302464 ) ) ;
#67441=CONICAL_SURFACE ( 'NONE', #27761, 0.1000000000000000472, 0.003490658503988666988 ) ;
#67442=ORIENTED_EDGE ( 'NONE', *, *, #128425, .T. ) ;
#67443=CARTESIAN_POINT ( 'NONE',  ( -2.950000000000030376, 2.500000000000000000, 6.495190528383297135 ) ) ;
#67445=VERTEX_POINT ( 'NONE', #68009 ) ;
#67446=EDGE_CURVE ( 'NONE', #61230, #96281, #18266, .T. ) ;
#67447=DIRECTION ( 'NONE',  ( 0.000000000000000000, 0.000000000000000000, -1.000000000000000000 ) ) ;
#67448=CONICAL_SURFACE ( 'NONE', #90558, 0.1000000000000002554, 0.003490658503988666988 ) ;
#67449=EDGE_CURVE ( 'NONE', #120047, #66944, #17655, .T. ) ;
#67450=ORIENTED_EDGE ( 'NONE', *, *, #99395, .T. ) ;
#67451=CARTESIAN_POINT ( 'NONE',  ( 6.649999999999930189, 2.500000000000000000, 7.288010851410849256 ) ) ;
#67452=DIRECTION ( 'NONE',  ( -0.000000000000000000, 1.000000000000000000, -0.000000000000000000 ) ) ;
#67453=ADVANCED_FACE ( 'NONE', ( #18901 ), #71896, .T. ) ;
#67454=CARTESIAN_POINT ( 'NONE',  ( 7.899999999999924860, 2.500000000000000000, -3.637306695894650055 ) ) ;
#67455=EDGE_CURVE ( 'NONE', #122964, #56169, #2476, .T. ) ;
#67456=DIRECTION ( 'NONE',  ( 0.000000000000000000, -0.9999939076577903929, 0.003490651415223739937 ) ) ;
#67457=ORIENTED_EDGE ( 'NONE', *, *, #115906, .T. ) ;
#67458=DIRECTION ( 'NONE',  ( -4.274815082592931898E-19, -0.9999939076577903929, -0.003490651415223739937 ) ) ;
#67459=DIRECTION ( 'NONE',  ( 0.000000000000000000, 1.000000000000000000, 0.000000000000000000 ) ) ;
#67461=CARTESIAN_POINT ( 'NONE',  ( 3.299999999999944755, 2.500000000000000000, 0.09999999999999761857 ) ) ;
#67462=PLANE ( 'NONE',  #51570 ) ;
#67463=EDGE_CURVE ( 'NONE', #71667, #108330, #55236, .T. ) ;
#67464=AXIS2_PLACEMENT_3D ( 'NONE', #35711, #16682, #16042 ) ;
#67465=ORIENTED_EDGE ( 'NONE', *, *, #106873, .T. ) ;
#67466=EDGE_LOOP ( 'NONE', ( #57811, #4080, #62653, #89555 ) ) ;
#67467=DIRECTION ( 'NONE',  ( 0.000000000000000000, 0.000000000000000000, 1.000000000000000000 ) ) ;
#67468=EDGE_LOOP ( 'NONE', ( #93958, #45804, #112693, #34745 ) ) ;
#67469=PLANE ( 'NONE',  #59783 ) ;
#67470=ORIENTED_EDGE ( 'NONE', *, *, #123164, .T. ) ;
#67471=ORIENTED_EDGE ( 'NONE', *, *, #126328, .T. ) ;
#67472=ORIENTED_EDGE ( 'NONE', *, *, #13506, .T. ) ;
#67473=DIRECTION ( 'NONE',  ( 0.000000000000000000, 1.000000000000000000, 0.000000000000000000 ) ) ;
#67474=AXIS2_PLACEMENT_3D ( 'NONE', #124109, #65172, #34465 ) ;
#67475=CARTESIAN_POINT ( 'NONE',  ( -9.400000000000009237, 2.500000000000000000, -4.083716857408422385 ) ) ;
#67476=CIRCLE ( 'NONE', #27783, 0.1000000000000002554 ) ;
#67477=DIRECTION ( 'NONE',  ( -0.000000000000000000, 1.000000000000000000, -0.000000000000000000 ) ) ;
#67479=CARTESIAN_POINT ( 'NONE',  ( -8.150000000000014566, 2.500000000000000000, -6.148780366869520897 ) ) ;
#67480=CARTESIAN_POINT ( 'NONE',  ( -9.600000000000006750, 2.500000000000000000, 0.5928203230275495006 ) ) ;
#67481=CARTESIAN_POINT ( 'NONE',  ( 12.69999999999990159, 2.500000000000000000, 4.676537180435972552 ) ) ;
#67482=FACE_OUTER_BOUND ( 'NONE', #40058, .T. ) ;
#67483=EDGE_CURVE ( 'NONE', #128073, #77956, #23939, .T. ) ;
#67484=ORIENTED_EDGE ( 'NONE', *, *, #86997, .F. ) ;
#67485=AXIS2_PLACEMENT_3D ( 'NONE', #105436, #15744, #95612 ) ;
#67486=AXIS2_PLACEMENT_3D ( 'NONE', #123853, #35501, #15175 ) ;
#67487=FACE_OUTER_BOUND ( 'NONE', #104974, .T. ) ;
#67488=EDGE_LOOP ( 'NONE', ( #59156, #110097, #94003, #128152 ) ) ;
#67489=AXIS2_PLACEMENT_3D ( 'NONE', #58960, #108049, #98226 ) ;
#67490=ORIENTED_EDGE ( 'NONE', *, *, #109998, .T. ) ;
#67491=ORIENTED_EDGE ( 'NONE', *, *, #65848, .F. ) ;
#67493=CARTESIAN_POINT ( 'NONE',  ( -12.49999999999999467, 12.50000000000000000, 0.7579135962115910452 ) ) ;
#67494=ORIENTED_EDGE ( 'NONE', *, *, #75683, .F. ) ;
#67495=ORIENTED_EDGE ( 'NONE', *, *, #119132, .F. ) ;
#67496=CONICAL_SURFACE ( 'NONE', #25751, 0.09999999999999982514, 0.003490658503988666988 ) ;
#67497=AXIS2_PLACEMENT_3D ( 'NONE', #80283, #120205, #70456 ) ;
#67498=DIRECTION ( 'NONE',  ( -0.000000000000000000, -1.000000000000000000, -0.000000000000000000 ) ) ;
#67499=CARTESIAN_POINT ( 'NONE',  ( -3.749999999999991118, 12.50000000000000000, -2.165063509461101710 ) ) ;
#67500=ADVANCED_FACE ( 'NONE', ( #1842 ), #111818, .T. ) ;
#67501=DIRECTION ( 'NONE',  ( 0.000000000000000000, 0.000000000000000000, 1.000000000000000000 ) ) ;
#67502=AXIS2_PLACEMENT_3D ( 'NONE', #30678, #127568, #88935 ) ;
#67503=DIRECTION ( 'NONE',  ( 0.000000000000000000, 0.000000000000000000, -1.000000000000000000 ) ) ;
#67504=AXIS2_PLACEMENT_3D ( 'NONE', #9086, #85707, #125625 ) ;
#67505=AXIS2_PLACEMENT_3D ( 'NONE', #47063, #56844, #28710 ) ;
#67506=FACE_OUTER_BOUND ( 'NONE', #78780, .T. ) ;
#67507=EDGE_LOOP ( 'NONE', ( #4821, #73278 ) ) ;
#67508=CONICAL_SURFACE ( 'NONE', #6857, 0.09999999999999982514, 0.003490658503988666988 ) ;
#67509=CARTESIAN_POINT ( 'NONE',  ( -0.2000000000000408673, 12.50000000000000000, -3.918623584224389056 ) ) ;
#67510=ORIENTED_EDGE ( 'NONE', *, *, #115500, .F. ) ;
#67511=DIRECTION ( 'NONE',  ( -4.274815082592931898E-19, -0.9999939076577903929, -0.003490651415223739937 ) ) ;
#67512=ORIENTED_EDGE ( 'NONE', *, *, #12144, .F. ) ;
#67513=AXIS2_PLACEMENT_3D ( 'NONE', #128846, #88208, #67269 ) ;
#67514=CARTESIAN_POINT ( 'NONE',  ( 7.049999999999928768, 12.50000000000000000, -2.099970236277064473 ) ) ;
#67515=ORIENTED_EDGE ( 'NONE', *, *, #98816, .F. ) ;
#67516=EDGE_CURVE ( 'NONE', #97603, #33814, #107552, .T. ) ;
#67517=ORIENTED_EDGE ( 'NONE', *, *, #45984, .T. ) ;
#67518=FACE_OUTER_BOUND ( 'NONE', #2228, .T. ) ;
#67519=DIRECTION ( 'NONE',  ( 0.000000000000000000, -0.000000000000000000, 1.000000000000000000 ) ) ;
#67520=CARTESIAN_POINT ( 'NONE',  ( -5.600000000000020073, 12.50000000000000000, 3.983716857408420964 ) ) ;
#67521=FACE_OUTER_BOUND ( 'NONE', #41082, .T. ) ;
#67522=B_SPLINE_CURVE_WITH_KNOTS ( 'NONE', 3,
 ( #39711, #10832, #373, #91999, #50157, #60624, #89420, #91349, #121445, #21314 ),
 .UNSPECIFIED., .F., .F.,
 ( 4, 2, 2, 2, 4 ),
 ( -0.0001133383185231292639, 0.01648990952740256311, 0.03309315737332825524, 0.04969640521925394738, 0.06629965306517963952 ),
 .UNSPECIFIED. ) ;
#67523=CARTESIAN_POINT ( 'NONE',  ( -15.79999999999998117, 2.500000000000000000, -0.1000000000000000056 ) ) ;
#67524=EDGE_LOOP ( 'NONE', ( #48500, #107212, #119978, #90763 ) ) ;
#67525=CARTESIAN_POINT ( 'NONE',  ( 4.399999999999939071, 12.50000000000000000, -0.3464101615137782364 ) ) ;
#67526=DIRECTION ( 'NONE',  ( 0.000000000000000000, 0.000000000000000000, 1.000000000000000000 ) ) ;
#67527=AXIS2_PLACEMENT_3D ( 'NONE', #41293, #30835, #40660 ) ;
#67528=AXIS2_PLACEMENT_3D ( 'NONE', #29414, #70617, #81095 ) ;
#67529=DIRECTION ( 'NONE',  ( -0.000000000000000000, 1.000000000000000000, -0.000000000000000000 ) ) ;
#67530=FACE_OUTER_BOUND ( 'NONE', #13669, .T. ) ;
#67531=FACE_OUTER_BOUND ( 'NONE', #37306, .T. ) ;
#67532=ORIENTED_EDGE ( 'NONE', *, *, #22733, .T. ) ;
#67533=CONICAL_SURFACE ( 'NONE', #107263, 0.1000000000000002554, 0.003490658503988666988 ) ;
#67534=AXIS2_PLACEMENT_3D ( 'NONE', #69381, #18353, #99511 ) ;
#67537=CIRCLE ( 'NONE', #94746, 0.06509327318403745899 ) ;
#67538=CARTESIAN_POINT ( 'NONE',  ( 2.049999999999950084, 2.500000000000000000, -6.495190528383302464 ) ) ;
#67539=ORIENTED_EDGE ( 'NONE', *, *, #20882, .F. ) ;
#67540=CARTESIAN_POINT ( 'NONE',  ( 14.34999999999989662, 2.500000000000000000, 2.411473670974873862 ) ) ;
#67541=DIRECTION ( 'NONE',  ( 0.000000000000000000, 1.000000000000000000, 0.000000000000000000 ) ) ;
#67542=VECTOR ( 'NONE', #57560, 1000.000000000000000 ) ;
#67543=VECTOR ( 'NONE', #60022, 1000.000000000000000 ) ;
#67544=AXIS2_PLACEMENT_3D ( 'NONE', #42800, #80770, #3484 ) ;
#67545=EDGE_CURVE ( 'NONE', #69354, #18837, #42435, .T. ) ;
#67546=AXIS2_PLACEMENT_3D ( 'NONE', #73770, #3747, #122890 ) ;
#67547=AXIS2_PLACEMENT_3D ( 'NONE', #89108, #87159, #77355 ) ;
#67548=ORIENTED_EDGE ( 'NONE', *, *, #100030, .T. ) ;
#67550=CARTESIAN_POINT ( 'NONE',  ( 10.59999999999990905, 2.500000000000000000, 4.083716857408420609 ) ) ;
#67551=DIRECTION ( 'NONE',  ( 0.000000000000000000, 0.000000000000000000, 1.000000000000000000 ) ) ;
#67552=CARTESIAN_POINT ( 'NONE',  ( 14.14999999999989377, 12.50000000000000000, -1.472243186433550122 ) ) ;
#67553=EDGE_LOOP ( 'NONE', ( #91649, #44374 ) ) ;
#67555=EDGE_CURVE ( 'NONE', #46396, #108554, #97084, .T. ) ;
#67556=DIRECTION ( 'NONE',  ( 0.000000000000000000, 1.000000000000000000, 0.000000000000000000 ) ) ;
#67557=DIRECTION ( 'NONE',  ( -0.000000000000000000, 1.000000000000000000, -0.000000000000000000 ) ) ;
#67558=ORIENTED_EDGE ( 'NONE', *, *, #31029, .F. ) ;
#67559=EDGE_CURVE ( 'NONE', #15257, #58594, #81694, .T. ) ;
#67560=EDGE_CURVE ( 'NONE', #59645, #125100, #31332, .T. ) ;
#67562=CARTESIAN_POINT ( 'NONE',  ( -1.900000000000034106, 2.500000000000000000, -4.083716857408426826 ) ) ;
#67563=EDGE_CURVE ( 'NONE', #125412, #6322, #101352, .T. ) ;
#67564=CARTESIAN_POINT ( 'NONE',  ( 6.849999999999927702, 12.50000000000000000, 1.818653347947321475 ) ) ;
#67565=DIRECTION ( 'NONE',  ( 0.000000000000000000, 0.000000000000000000, 1.000000000000000000 ) ) ;
#67566=CIRCLE ( 'NONE', #71800, 0.09999999999999999167 ) ;
#67567=EDGE_LOOP ( 'NONE', ( #99416, #32634 ) ) ;
#67568=DIRECTION ( 'NONE',  ( 0.000000000000000000, 1.000000000000000000, 0.000000000000000000 ) ) ;
#67569=ORIENTED_EDGE ( 'NONE', *, *, #77912, .T. ) ;
#67570=DIRECTION ( 'NONE',  ( 0.000000000000000000, -0.000000000000000000, 1.000000000000000000 ) ) ;
#67571=DIRECTION ( 'NONE',  ( 0.000000000000000000, 0.000000000000000000, 1.000000000000000000 ) ) ;
#67572=EDGE_CURVE ( 'NONE', #54801, #120522, #30209, .T. ) ;
#67573=DIRECTION ( 'NONE',  ( -0.000000000000000000, 1.000000000000000000, -0.000000000000000000 ) ) ;
#67574=AXIS2_PLACEMENT_3D ( 'NONE', #26047, #13631, #3195 ) ;
#67575=VERTEX_POINT ( 'NONE', #100059 ) ;
#67576=AXIS2_PLACEMENT_3D ( 'NONE', #34316, #74869, #95151 ) ;
#67577=EDGE_CURVE ( 'NONE', #25440, #39251, #120081, .T. ) ;
#67578=CIRCLE ( 'NONE', #48738, 0.1000000000000000472 ) ;
#67579=CARTESIAN_POINT ( 'NONE',  ( -12.04999999999999538, 12.50000000000000000, 6.495190528383297135 ) ) ;
#67580=ADVANCED_FACE ( 'NONE', ( #10383 ), #28138, .T. ) ;
#67581=DIRECTION ( 'NONE',  ( 0.000000000000000000, 1.000000000000000000, 0.000000000000000000 ) ) ;
#67582=ORIENTED_EDGE ( 'NONE', *, *, #80130, .T. ) ;
#67583=DIRECTION ( 'NONE',  ( -4.274815082592931898E-19, -0.9999939076577903929, -0.003490651415223739937 ) ) ;
#67584=AXIS2_PLACEMENT_3D ( 'NONE', #1274, #30760, #129609 ) ;
#67585=ORIENTED_EDGE ( 'NONE', *, *, #51074, .F. ) ;
#67586=AXIS2_PLACEMENT_3D ( 'NONE', #83639, #20846, #62071 ) ;
#67587=CARTESIAN_POINT ( 'NONE',  ( -9.150000000000009237, 12.50000000000000000, 1.472243186433545459 ) ) ;
#67588=AXIS2_PLACEMENT_3D ( 'NONE', #88748, #8241, #116897 ) ;
#67589=AXIS2_PLACEMENT_3D ( 'NONE', #52128, #20088, #91392 ) ;
#67590=ORIENTED_EDGE ( 'NONE', *, *, #93787, .T. ) ;
#67591=DIRECTION ( 'NONE',  ( 0.000000000000000000, 1.000000000000000000, 0.000000000000000000 ) ) ;
#67592=DIRECTION ( 'NONE',  ( 0.000000000000000000, 0.000000000000000000, 1.000000000000000000 ) ) ;
#67594=ORIENTED_EDGE ( 'NONE', *, *, #33258, .T. ) ;
#67595=VECTOR ( 'NONE', #14177, 1000.000000000000000 ) ;
#67596=DIRECTION ( 'NONE',  ( 0.000000000000000000, -0.9999939076577903929, 0.003490651415223739937 ) ) ;
#67597=LINE ( 'NONE', #86598, #75641 ) ;
#67599=CARTESIAN_POINT ( 'NONE',  ( -10.40000000000000213, 2.500000000000000000, -0.6928203230275541413 ) ) ;
#67600=DIRECTION ( 'NONE',  ( -0.000000000000000000, 1.000000000000000000, -0.000000000000000000 ) ) ;
#67601=AXIS2_PLACEMENT_3D ( 'NONE', #30429, #117454, #99795 ) ;
#67602=CONICAL_SURFACE ( 'NONE', #11176, 0.1000000000000000056, 0.003490658503988666988 ) ;
#67603=VECTOR ( 'NONE', #118858, 1000.000000000000000 ) ;
#67604=DIRECTION ( 'NONE',  ( -0.000000000000000000, -1.000000000000000000, -0.000000000000000000 ) ) ;
#67605=CARTESIAN_POINT ( 'NONE',  ( 3.099999999999945022, 2.500000000000000000, -4.776537180435978414 ) ) ;
#67607=FACE_OUTER_BOUND ( 'NONE', #22289, .T. ) ;
#67608=ORIENTED_EDGE ( 'NONE', *, *, #115570, .F. ) ;
#67609=ORIENTED_EDGE ( 'NONE', *, *, #20947, .T. ) ;
#67610=VERTEX_POINT ( 'NONE', #80426 ) ;
#67611=ORIENTED_EDGE ( 'NONE', *, *, #3513, .F. ) ;
#67612=LINE ( 'NONE', #66333, #72609 ) ;
#67613=CARTESIAN_POINT ( 'NONE',  ( 9.349999999999916156, 2.500000000000000000, 6.841600689897072485 ) ) ;
#67614=DIRECTION ( 'NONE',  ( -0.000000000000000000, -1.000000000000000000, -0.000000000000000000 ) ) ;
#67615=ORIENTED_EDGE ( 'NONE', *, *, #54700, .T. ) ;
#67616=FACE_BOUND ( 'NONE', #74253, .T. ) ;
#67617=ORIENTED_EDGE ( 'NONE', *, *, #129605, .F. ) ;
#67618=EDGE_CURVE ( 'NONE', #92344, #118717, #32638, .T. ) ;
#67619=PLANE ( 'NONE',  #35475 ) ;
#67620=DIRECTION ( 'NONE',  ( 0.000000000000000000, -0.9999939076577903929, 0.003490651415223739937 ) ) ;
#67621=EDGE_CURVE ( 'NONE', #20397, #97989, #128417, .T. ) ;
#67622=CARTESIAN_POINT ( 'NONE',  ( 87.50000000000001421, 0.000000000000000000, 0.000000000000000000 ) ) ;
#67623=DIRECTION ( 'NONE',  ( -0.000000000000000000, 1.000000000000000000, -0.000000000000000000 ) ) ;
#67624=EDGE_CURVE ( 'NONE', #91497, #15344, #32275, .T. ) ;
#67625=CARTESIAN_POINT ( 'NONE',  ( 16.32066102237043737, -2.500000000000000000, 4.877377760480507085 ) ) ;
#67626=LINE ( 'NONE', #85971, #10030 ) ;
#67627=DIRECTION ( 'NONE',  ( 0.000000000000000000, 1.000000000000000000, 0.000000000000000000 ) ) ;
#67628=CARTESIAN_POINT ( 'NONE',  ( 10.39999999999991154, 2.500000000000000000, 3.737306695894644371 ) ) ;
#67629=AXIS2_PLACEMENT_3D ( 'NONE', #53035, #44492, #43231 ) ;
#67630=AXIS2_PLACEMENT_3D ( 'NONE', #20232, #99449, #129571 ) ;
#67631=CARTESIAN_POINT ( 'NONE',  ( -1.050000000000038680, 2.500000000000000000, 2.611473670974873151 ) ) ;
#67632=DIRECTION ( 'NONE',  ( 0.000000000000000000, 0.000000000000000000, 1.000000000000000000 ) ) ;
#67633=EDGE_CURVE ( 'NONE', #106590, #106830, #122146, .T. ) ;
#67634=AXIS2_PLACEMENT_3D ( 'NONE', #99146, #42151, #31687 ) ;
#67635=CONICAL_SURFACE ( 'NONE', #46722, 0.09999999999999982514, 0.003490658503988666988 ) ;
#67636=ORIENTED_EDGE ( 'NONE', *, *, #42685, .T. ) ;
#67637=ORIENTED_EDGE ( 'NONE', *, *, #56224, .F. ) ;
#67638=ORIENTED_EDGE ( 'NONE', *, *, #34660, .F. ) ;
#67639=AXIS2_PLACEMENT_3D ( 'NONE', #44441, #84364, #124296 ) ;
#67640=ORIENTED_EDGE ( 'NONE', *, *, #27569, .F. ) ;
#67641=CARTESIAN_POINT ( 'NONE',  ( 16.73289298692360205, -0.7002450284381240841, -5.897165230078514675 ) ) ;
#67642=AXIS2_PLACEMENT_3D ( 'NONE', #23373, #72504, #82321 ) ;
#67643=CARTESIAN_POINT ( 'NONE',  ( -11.84999999999999609, 2.500000000000000000, 6.048780366869521252 ) ) ;
#67644=EDGE_LOOP ( 'NONE', ( #11360, #60414, #2032, #49077 ) ) ;
#67645=ORIENTED_EDGE ( 'NONE', *, *, #15962, .T. ) ;
#67646=ORIENTED_EDGE ( 'NONE', *, *, #78717, .T. ) ;
#67648=AXIS2_PLACEMENT_3D ( 'NONE', #72088, #112008, #121172 ) ;
#67649=AXIS2_PLACEMENT_3D ( 'NONE', #127866, #192, #89235 ) ;
#67650=AXIS2_PLACEMENT_3D ( 'NONE', #104318, #97715, #80669 ) ;
#67651=PLANE ( 'NONE',  #56055 ) ;
#67652=DIRECTION ( 'NONE',  ( 0.000000000000000000, 1.000000000000000000, 0.000000000000000000 ) ) ;
#67653=DIRECTION ( 'NONE',  ( -0.000000000000000000, 1.000000000000000000, -0.000000000000000000 ) ) ;
#67654=DIRECTION ( 'NONE',  ( 0.000000000000000000, 1.000000000000000000, 0.000000000000000000 ) ) ;
#67655=VECTOR ( 'NONE', #76555, 1000.000000000000000 ) ;
#67656=DIRECTION ( 'NONE',  ( 0.000000000000000000, 0.000000000000000000, 1.000000000000000000 ) ) ;
#67657=EDGE_CURVE ( 'NONE', #95313, #115297, #13543, .T. ) ;
#67658=ORIENTED_EDGE ( 'NONE', *, *, #49920, .F. ) ;
#67659=CARTESIAN_POINT ( 'NONE',  ( -10.84999999999999964, 12.50000000000000000, 5.802370205355744659 ) ) ;
#67660=ORIENTED_EDGE ( 'NONE', *, *, #80124, .F. ) ;
#67661=VERTEX_POINT ( 'NONE', #75734 ) ;
#67662=ORIENTED_EDGE ( 'NONE', *, *, #33871, .T. ) ;
#67663=DIRECTION ( 'NONE',  ( 0.000000000000000000, 0.000000000000000000, -1.000000000000000000 ) ) ;
#67664=EDGE_LOOP ( 'NONE', ( #64222, #51714, #50274, #117383 ) ) ;
#67665=ORIENTED_EDGE ( 'NONE', *, *, #120914, .T. ) ;
#67666=CIRCLE ( 'NONE', #32197, 0.06509327318403745899 ) ;
#67667=LINE ( 'NONE', #118711, #12929 ) ;
#67668=DIRECTION ( 'NONE',  ( -0.000000000000000000, 1.000000000000000000, -0.000000000000000000 ) ) ;
#67669=DIRECTION ( 'NONE',  ( -4.274815082592931898E-19, -0.9999939076577903929, -0.003490651415223739937 ) ) ;
#67670=EDGE_CURVE ( 'NONE', #31226, #3120, #7280, .T. ) ;
#67672=PLANE ( 'NONE',  #16219 ) ;
#67673=AXIS2_PLACEMENT_3D ( 'NONE', #122168, #79646, #61310 ) ;
#67675=DIRECTION ( 'NONE',  ( 0.000000000000000000, 0.000000000000000000, -1.000000000000000000 ) ) ;
#67676=AXIS2_PLACEMENT_3D ( 'NONE', #62951, #70841, #31567 ) ;
#67677=CIRCLE ( 'NONE', #34261, 0.06509327318403745899 ) ;
#67678=VERTEX_POINT ( 'NONE', #54183 ) ;
#67679=DIRECTION ( 'NONE',  ( 0.000000000000000000, 0.000000000000000000, 1.000000000000000000 ) ) ;
#67680=EDGE_LOOP ( 'NONE', ( #51556, #42129, #128423, #71351 ) ) ;
#67682=DIRECTION ( 'NONE',  ( 0.000000000000000000, 0.000000000000000000, -1.000000000000000000 ) ) ;
#67683=ORIENTED_EDGE ( 'NONE', *, *, #61871, .T. ) ;
#67684=DIRECTION ( 'NONE',  ( -4.274815082592931898E-19, -0.9999939076577903929, -0.003490651415223739937 ) ) ;
#67685=ADVANCED_FACE ( 'NONE', ( #93454 ), #59562, .T. ) ;
#67686=DIRECTION ( 'NONE',  ( 0.000000000000000000, -0.9999939076577903929, 0.003490651415223739937 ) ) ;
#67687=CONICAL_SURFACE ( 'NONE', #36415, 0.1000000000000002554, 0.003490658503988666988 ) ;
#67689=CIRCLE ( 'NONE', #17196, 0.09999999999999982514 ) ;
#67690=AXIS2_PLACEMENT_3D ( 'NONE', #104437, #43604, #103800 ) ;
#67691=LINE ( 'NONE', #108270, #113531 ) ;
#67692=EDGE_LOOP ( 'NONE', ( #35360, #29536 ) ) ;
#67693=EDGE_CURVE ( 'NONE', #67035, #97177, #95130, .T. ) ;
#67694=VERTEX_POINT ( 'NONE', #113751 ) ;
#67695=PLANE ( 'NONE',  #1672 ) ;
#67696=CARTESIAN_POINT ( 'NONE',  ( -0.4000000000000331624, 2.500000000000000000, -0.1000000000000000056 ) ) ;
#67698=AXIS2_PLACEMENT_3D ( 'NONE', #28533, #336, #9538 ) ;
#67699=CARTESIAN_POINT ( 'NONE',  ( -5.000000000000023093, 12.50000000000000000, 0.7579135962115869374 ) ) ;
#67700=CARTESIAN_POINT ( 'NONE',  ( -5.600000000000020073, 2.500000000000000000, 0.3464101615137736845 ) ) ;
#67701=CIRCLE ( 'NONE', #61471, 0.1000000000000002554 ) ;
#67702=VECTOR ( 'NONE', #11993, 1000.000000000000000 ) ;
#67703=AXIS2_PLACEMENT_3D ( 'NONE', #88515, #69524, #78730 ) ;
#67704=DIRECTION ( 'NONE',  ( 0.000000000000000000, 0.000000000000000000, 1.000000000000000000 ) ) ;
#67705=AXIS2_PLACEMENT_3D ( 'NONE', #27067, #118656, #159 ) ;
#67706=ORIENTED_EDGE ( 'NONE', *, *, #97464, .F. ) ;
#67707=DIRECTION ( 'NONE',  ( 0.000000000000000000, 1.000000000000000000, 0.000000000000000000 ) ) ;
#67708=LINE ( 'NONE', #48088, #14445 ) ;
#67709=EDGE_CURVE ( 'NONE', #11527, #99935, #42835, .T. ) ;
#67710=VERTEX_POINT ( 'NONE', #96030 ) ;
#67711=DIRECTION ( 'NONE',  ( 0.000000000000000000, 0.000000000000000000, 1.000000000000000000 ) ) ;
#67713=CARTESIAN_POINT ( 'NONE',  ( -8.750000000000008882, 12.50000000000000000, -2.922977105672691422 ) ) ;
#67714=DIRECTION ( 'NONE',  ( 0.000000000000000000, 0.000000000000000000, 1.000000000000000000 ) ) ;
#67715=DIRECTION ( 'NONE',  ( 0.000000000000000000, 1.000000000000000000, 0.000000000000000000 ) ) ;
#67716=ORIENTED_EDGE ( 'NONE', *, *, #49588, .T. ) ;
#67717=EDGE_CURVE ( 'NONE', #60832, #26300, #14859, .T. ) ;
#67718=DIRECTION ( 'NONE',  ( -0.000000000000000000, 1.000000000000000000, -0.000000000000000000 ) ) ;
#67719=CARTESIAN_POINT ( 'NONE',  ( 6.899999999999928413, 12.50000000000000000, -4.676537180435977881 ) ) ;
#67720=AXIS2_PLACEMENT_3D ( 'NONE', #61756, #218, #40174 ) ;
#67721=AXIS2_PLACEMENT_3D ( 'NONE', #5047, #26636, #56083 ) ;
#67722=EDGE_CURVE ( 'NONE', #87229, #23494, #40769, .T. ) ;
#67723=AXIS2_PLACEMENT_3D ( 'NONE', #71996, #51710, #43191 ) ;
#67724=ADVANCED_FACE ( 'NONE', ( #45656 ), #65264, .T. ) ;
#67725=EDGE_CURVE ( 'NONE', #125960, #56674, #109712, .T. ) ;
#67727=ORIENTED_EDGE ( 'NONE', *, *, #79718, .F. ) ;
#67728=DIRECTION ( 'NONE',  ( -0.000000000000000000, 1.000000000000000000, -0.000000000000000000 ) ) ;
#67729=VECTOR ( 'NONE', #117966, 1000.000000000000000 ) ;
#67730=AXIS2_PLACEMENT_3D ( 'NONE', #99914, #118899, #80274 ) ;
#67732=AXIS2_PLACEMENT_3D ( 'NONE', #19925, #121329, #72885 ) ;
#67733=ORIENTED_EDGE ( 'NONE', *, *, #65325, .T. ) ;
#67735=ADVANCED_FACE ( 'NONE', ( #44346 ), #34507, .T. ) ;
#67736=EDGE_CURVE ( 'NONE', #20628, #126381, #101392, .T. ) ;
#67738=LINE ( 'NONE', #6859, #117545 ) ;
#67739=CARTESIAN_POINT ( 'NONE',  ( 13.14999999999990088, 12.50000000000000000, 1.818653347947321475 ) ) ;
#67740=ADVANCED_FACE ( 'NONE', ( #124851 ), #24720, .T. ) ;
#67741=DIRECTION ( 'NONE',  ( -0.000000000000000000, -1.000000000000000000, -0.000000000000000000 ) ) ;
#67742=VECTOR ( 'NONE', #115695, 1000.000000000000000 ) ;
#67743=ORIENTED_EDGE ( 'NONE', *, *, #87871, .T. ) ;
#67744=EDGE_CURVE ( 'NONE', #9132, #94097, #36560, .T. ) ;
#67745=AXIS2_PLACEMENT_3D ( 'NONE', #5989, #67477, #25005 ) ;
#67746=CONICAL_SURFACE ( 'NONE', #11318, 0.09999999999999982514, 0.003490658503988666988 ) ;
#67747=FACE_OUTER_BOUND ( 'NONE', #46483, .T. ) ;
#67748=EDGE_CURVE ( 'NONE', #12970, #120897, #61687, .T. ) ;
#67749=DIRECTION ( 'NONE',  ( 0.000000000000000000, 0.000000000000000000, 1.000000000000000000 ) ) ;
#67750=ORIENTED_EDGE ( 'NONE', *, *, #111511, .T. ) ;
#67751=AXIS2_PLACEMENT_3D ( 'NONE', #101360, #39873, #79775 ) ;
#67752=CARTESIAN_POINT ( 'NONE',  ( -3.300000000000028244, 12.50000000000000000, 4.330127018922196314 ) ) ;
#67753=CARTESIAN_POINT ( 'NONE',  ( -1.050000000000037792, 12.50000000000000000, 1.818653347947321475 ) ) ;
#67754=ADVANCED_FACE ( 'NONE', ( #35824 ), #24029, .T. ) ;
#67755=EDGE_LOOP ( 'NONE', ( #73320, #9002, #9032, #120132 ) ) ;
#67756=VERTEX_POINT ( 'NONE', #103284 ) ;
#67757=VERTEX_POINT ( 'NONE', #122926 ) ;
#67758=PLANE ( 'NONE',  #16941 ) ;
#67759=CIRCLE ( 'NONE', #17276, 0.06509327318403745899 ) ;
#67760=DIRECTION ( 'NONE',  ( 0.000000000000000000, 1.000000000000000000, 0.000000000000000000 ) ) ;
#67761=DIRECTION ( 'NONE',  ( -4.274815082592931898E-19, -0.9999939076577903929, -0.003490651415223739937 ) ) ;
#67762=FACE_BOUND ( 'NONE', #10393, .T. ) ;
#67763=ORIENTED_EDGE ( 'NONE', *, *, #127538, .T. ) ;
#67764=CARTESIAN_POINT ( 'NONE',  ( 4.999999999999969802, 2.500000000000000000, 4.230127018922196669 ) ) ;
#67766=CIRCLE ( 'NONE', #11339, 0.06509327318403745899 ) ;
#67767=ORIENTED_EDGE ( 'NONE', *, *, #23658, .F. ) ;
#67768=DIRECTION ( 'NONE',  ( 0.000000000000000000, 1.000000000000000000, 0.000000000000000000 ) ) ;
#67769=CARTESIAN_POINT ( 'NONE',  ( -12.09999999999999609, 12.50000000000000000, 4.265033745738159077 ) ) ;
#67770=DIRECTION ( 'NONE',  ( 0.000000000000000000, 1.000000000000000000, 0.000000000000000000 ) ) ;
#67771=DIRECTION ( 'NONE',  ( 0.000000000000000000, 1.000000000000000000, 0.000000000000000000 ) ) ;
#67772=DIRECTION ( 'NONE',  ( -0.000000000000000000, 1.000000000000000000, -0.000000000000000000 ) ) ;
#67773=CIRCLE ( 'NONE', #17590, 0.06509327318403745899 ) ;
#67774=AXIS2_PLACEMENT_3D ( 'NONE', #122500, #11887, #73382 ) ;
#67775=ORIENTED_EDGE ( 'NONE', *, *, #113346, .T. ) ;
#67776=ORIENTED_EDGE ( 'NONE', *, *, #125367, .T. ) ;
#67777=EDGE_LOOP ( 'NONE', ( #71152, #127580, #105516, #23490 ) ) ;
#67778=VERTEX_POINT ( 'NONE', #83644 ) ;
#67779=ORIENTED_EDGE ( 'NONE', *, *, #105190, .T. ) ;
#67780=CARTESIAN_POINT ( 'NONE',  ( 0.1999999999999576006, 2.500000000000000000, -4.676537180435978769 ) ) ;
#67781=CARTESIAN_POINT ( 'NONE',  ( -12.29999999999999361, 2.500000000000000000, 3.883716857408420431 ) ) ;
#67782=ORIENTED_EDGE ( 'NONE', *, *, #87358, .T. ) ;
#67783=FACE_BOUND ( 'NONE', #29609, .T. ) ;
#67784=DIRECTION ( 'NONE',  ( 0.000000000000000000, 0.000000000000000000, -1.000000000000000000 ) ) ;
#67785=AXIS2_PLACEMENT_3D ( 'NONE', #120066, #110241, #81434 ) ;
#67786=EDGE_CURVE ( 'NONE', #125792, #59408, #9348, .T. ) ;
#67787=DIRECTION ( 'NONE',  ( 0.000000000000000000, 0.000000000000000000, 1.000000000000000000 ) ) ;
#67788=EDGE_CURVE ( 'NONE', #101569, #116415, #128604, .T. ) ;
#67790=DIRECTION ( 'NONE',  ( 0.000000000000000000, 0.000000000000000000, 1.000000000000000000 ) ) ;
#67791=CARTESIAN_POINT ( 'NONE',  ( -3.750000000000029310, 2.500000000000000000, -7.188010851410854052 ) ) ;
#67792=ORIENTED_EDGE ( 'NONE', *, *, #64325, .T. ) ;
#67793=CARTESIAN_POINT ( 'NONE',  ( 16.98389447545005027, -2.500000000000469402, 5.627887033854102938 ) ) ;
#67794=EDGE_CURVE ( 'NONE', #62518, #36092, #126437, .T. ) ;
#67795=ORIENTED_EDGE ( 'NONE', *, *, #30509, .T. ) ;
#67796=AXIS2_PLACEMENT_3D ( 'NONE', #32208, #13163, #73385 ) ;
#67797=CIRCLE ( 'NONE', #40729, 0.1000000000000002554 ) ;
#67798=ORIENTED_EDGE ( 'NONE', *, *, #70124, .F. ) ;
#67799=ORIENTED_EDGE ( 'NONE', *, *, #117975, .F. ) ;
#67800=CARTESIAN_POINT ( 'NONE',  ( 97.50000000000000000, -1.500000000000000222, 1.322875655532295136 ) ) ;
#67801=DIRECTION ( 'NONE',  ( 0.000000000000000000, 0.000000000000000000, 1.000000000000000000 ) ) ;
#67802=DIRECTION ( 'NONE',  ( -0.000000000000000000, 1.000000000000000000, -0.000000000000000000 ) ) ;
#67803=AXIS2_PLACEMENT_3D ( 'NONE', #110133, #820, #40777 ) ;
#67804=ORIENTED_EDGE ( 'NONE', *, *, #60532, .T. ) ;
#67805=DIRECTION ( 'NONE',  ( 0.000000000000000000, 1.000000000000000000, 0.000000000000000000 ) ) ;
#67806=VECTOR ( 'NONE', #12838, 1000.000000000000000 ) ;
#67807=DIRECTION ( 'NONE',  ( -0.000000000000000000, -1.000000000000000000, -0.000000000000000000 ) ) ;
#67808=DIRECTION ( 'NONE',  ( 0.000000000000000000, 0.000000000000000000, 1.000000000000000000 ) ) ;
#67810=DIRECTION ( 'NONE',  ( 0.000000000000000000, 1.000000000000000000, 0.000000000000000000 ) ) ;
#67811=CARTESIAN_POINT ( 'NONE',  ( 7.899999999999924860, 12.50000000000000000, 4.395220292106234439 ) ) ;
#67812=CARTESIAN_POINT ( 'NONE',  ( -11.64999999999999680, 2.500000000000000000, 1.472243186433545459 ) ) ;
#67813=ORIENTED_EDGE ( 'NONE', *, *, #11711, .F. ) ;
#67814=FACE_OUTER_BOUND ( 'NONE', #10892, .T. ) ;
#67815=ORIENTED_EDGE ( 'NONE', *, *, #18951, .T. ) ;
#67816=AXIS2_PLACEMENT_3D ( 'NONE', #13098, #102151, #3937 ) ;
#67817=VERTEX_POINT ( 'NONE', #19387 ) ;
#67818=DIRECTION ( 'NONE',  ( -0.000000000000000000, -1.000000000000000000, -0.000000000000000000 ) ) ;
#67819=CONICAL_SURFACE ( 'NONE', #11386, 0.1000000000000002554, 0.003490658503988666988 ) ;
#67820=DIRECTION ( 'NONE',  ( -0.000000000000000000, 1.000000000000000000, -0.000000000000000000 ) ) ;
#67821=AXIS2_PLACEMENT_3D ( 'NONE', #60101, #52193, #72489 ) ;
#67822=CARTESIAN_POINT ( 'NONE',  ( -6.850000000000013856, 12.50000000000000000, 6.148780366869520897 ) ) ;
#67823=ORIENTED_EDGE ( 'NONE', *, *, #74731, .T. ) ;
#67824=VERTEX_POINT ( 'NONE', #18105 ) ;
#67825=ADVANCED_FACE ( 'NONE', ( #36490 ), #68496, .T. ) ;
#67827=AXIS2_PLACEMENT_3D ( 'NONE', #120963, #58827, #98733 ) ;
#67828=AXIS2_PLACEMENT_3D ( 'NONE', #89698, #59624, #97580 ) ;
#67829=AXIS2_PLACEMENT_3D ( 'NONE', #42923, #82835, #122742 ) ;
#67831=CARTESIAN_POINT ( 'NONE',  ( 4.549999999999937650, 2.500000000000000000, 2.165063509461097713 ) ) ;
#67832=ORIENTED_EDGE ( 'NONE', *, *, #49932, .F. ) ;
#67833=ORIENTED_EDGE ( 'NONE', *, *, #7992, .F. ) ;
#67834=CARTESIAN_POINT ( 'NONE',  ( -0.6000000000000323963, 12.50000000000000000, 0.3464101615137759604 ) ) ;
#67835=EDGE_LOOP ( 'NONE', ( #76124, #100297 ) ) ;
#67836=DIRECTION ( 'NONE',  ( 0.000000000000000000, 0.000000000000000000, 1.000000000000000000 ) ) ;
#67837=CIRCLE ( 'NONE', #95041, 0.09999999999999982514 ) ;
#67838=CONICAL_SURFACE ( 'NONE', #44875, 0.09999999999999999167, 0.003490658503988666988 ) ;
#67839=FACE_OUTER_BOUND ( 'NONE', #90107, .T. ) ;
#67840=VERTEX_POINT ( 'NONE', #77667 ) ;
#67841=DIRECTION ( 'NONE',  ( 0.000000000000000000, 1.000000000000000000, 0.000000000000000000 ) ) ;
#67842=FACE_OUTER_BOUND ( 'NONE', #59402, .T. ) ;
#67843=LINE ( 'NONE', #77657, #51121 ) ;
#67844=AXIS2_PLACEMENT_3D ( 'NONE', #27941, #5708, #67860 ) ;
#67845=EDGE_CURVE ( 'NONE', #4262, #109253, #72063, .T. ) ;
#67846=FACE_OUTER_BOUND ( 'NONE', #54725, .T. ) ;
#67847=ORIENTED_EDGE ( 'NONE', *, *, #114105, .T. ) ;
#67848=CARTESIAN_POINT ( 'NONE',  ( 8.349999999999923261, 12.50000000000000000, -5.867463478539787225 ) ) ;
#67849=VERTEX_POINT ( 'NONE', #108421 ) ;
#67850=ORIENTED_EDGE ( 'NONE', *, *, #14902, .F. ) ;
#67851=EDGE_CURVE ( 'NONE', #57277, #25898, #5229, .T. ) ;
#67852=FACE_OUTER_BOUND ( 'NONE', #99655, .T. ) ;
#67853=LINE ( 'NONE', #69135, #78423 ) ;
#67854=DIRECTION ( 'NONE',  ( -4.274815082592931898E-19, -0.9999939076577903929, -0.003490651415223739937 ) ) ;
#67855=DIRECTION ( 'NONE',  ( -0.000000000000000000, -1.000000000000000000, -0.000000000000000000 ) ) ;
#67856=VECTOR ( 'NONE', #108422, 1000.000000000000000 ) ;
#67857=DIRECTION ( 'NONE',  ( -4.274815082592931898E-19, -0.9999939076577903929, -0.003490651415223739937 ) ) ;
#67858=CARTESIAN_POINT ( 'NONE',  ( -4.400000000000025224, 12.50000000000000000, -0.3464101615137783474 ) ) ;
#67859=DIRECTION ( 'NONE',  ( 0.000000000000000000, 0.000000000000000000, 1.000000000000000000 ) ) ;
#67860=DIRECTION ( 'NONE',  ( 0.000000000000000000, 0.000000000000000000, -1.000000000000000000 ) ) ;
#67861=DIRECTION ( 'NONE',  ( 0.000000000000000000, 1.000000000000000000, 0.000000000000000000 ) ) ;
#67862=CARTESIAN_POINT ( 'NONE',  ( 7.299999999999927880, 2.500000000000000000, 3.983716857408420964 ) ) ;
#67863=CIRCLE ( 'NONE', #61625, 0.06509327318403745899 ) ;
#67864=CIRCLE ( 'NONE', #126366, 0.06509327318403745899 ) ;
#67865=ORIENTED_EDGE ( 'NONE', *, *, #31123, .T. ) ;
#67866=DIRECTION ( 'NONE',  ( -0.000000000000000000, 1.000000000000000000, -0.000000000000000000 ) ) ;
#67867=DIRECTION ( 'NONE',  ( 0.000000000000000000, 1.000000000000000000, 0.000000000000000000 ) ) ;
#67868=DIRECTION ( 'NONE',  ( 0.000000000000000000, 1.000000000000000000, 0.000000000000000000 ) ) ;
#67869=CARTESIAN_POINT ( 'NONE',  ( -9.150000000000009237, 2.500000000000000000, 2.857883832488649301 ) ) ;
#67870=FACE_OUTER_BOUND ( 'NONE', #128721, .T. ) ;
#67871=EDGE_LOOP ( 'NONE', ( #69975, #25693, #91100, #55209 ) ) ;
#67872=CARTESIAN_POINT ( 'NONE',  ( -0.4500000000000402012, 12.50000000000000000, 6.495190528383297135 ) ) ;
#67873=AXIS2_PLACEMENT_3D ( 'NONE', #110719, #21050, #60368 ) ;
#67875=AXIS2_PLACEMENT_3D ( 'NONE', #19658, #108671, #59608 ) ;
#67876=CARTESIAN_POINT ( 'NONE',  ( -7.499999999999980460, 2.500000000000000000, -4.330127018922201643 ) ) ;
#67877=CARTESIAN_POINT ( 'NONE',  ( -1.650000000000035660, 2.500000000000000000, 2.857883832488649301 ) ) ;
#67878=ORIENTED_EDGE ( 'NONE', *, *, #104995, .T. ) ;
#67879=ADVANCED_FACE ( 'NONE', ( #98585 ), #118894, .T. ) ;
#67880=EDGE_CURVE ( 'NONE', #64666, #59157, #3101, .T. ) ;
#67881=ORIENTED_EDGE ( 'NONE', *, *, #127338, .T. ) ;
#67882=CONICAL_SURFACE ( 'NONE', #69961, 0.09999999999999982514, 0.003490658503988666988 ) ;
#67883=CIRCLE ( 'NONE', #1081, 0.1000000000000000056 ) ;
#67884=ORIENTED_EDGE ( 'NONE', *, *, #92005, .T. ) ;
#67885=ORIENTED_EDGE ( 'NONE', *, *, #86047, .T. ) ;
#67886=VERTEX_POINT ( 'NONE', #16794 ) ;
#67887=CARTESIAN_POINT ( 'NONE',  ( 6.249999999999934275, 2.500000000000000000, -7.188010851410854052 ) ) ;
#67888=EDGE_CURVE ( 'NONE', #86766, #66020, #67853, .T. ) ;
#67889=EDGE_CURVE ( 'NONE', #25677, #249, #51227, .T. ) ;
#67890=VECTOR ( 'NONE', #126398, 1000.000000000000000 ) ;
#67891=EDGE_CURVE ( 'NONE', #111766, #92201, #8920, .T. ) ;
#67892=CARTESIAN_POINT ( 'NONE',  ( -5.850000000000021849, 2.500000000000000000, -7.288010851410854585 ) ) ;
#67893=DIRECTION ( 'NONE',  ( 0.000000000000000000, -0.9999939076577903929, 0.003490651415223739937 ) ) ;
#67894=VECTOR ( 'NONE', #51370, 1000.000000000000000 ) ;
#67895=DIRECTION ( 'NONE',  ( 0.000000000000000000, 1.000000000000000000, 0.000000000000000000 ) ) ;
#67897=ADVANCED_FACE ( 'NONE', ( #128744 ), #128075, .T. ) ;
#67898=DIRECTION ( 'NONE',  ( 0.000000000000000000, 1.000000000000000000, 0.000000000000000000 ) ) ;
#67899=ORIENTED_EDGE ( 'NONE', *, *, #49599, .T. ) ;
#67900=CARTESIAN_POINT ( 'NONE',  ( 26.75237029040465941, -2.962322469584636409, -2.722363819586870015 ) ) ;
#67901=DIRECTION ( 'NONE',  ( -0.000000000000000000, 1.000000000000000000, -0.000000000000000000 ) ) ;
#67902=CARTESIAN_POINT ( 'NONE',  ( 21.15177371151419194, 2.593223176056360213, 4.151029080743461108 ) ) ;
#67903=CARTESIAN_POINT ( 'NONE',  ( -3.150000000000029665, 12.50000000000000000, 6.906693963081109722 ) ) ;
#67904=DIRECTION ( 'NONE',  ( -4.274815082592931898E-19, -0.9999939076577903929, -0.003490651415223739937 ) ) ;
#67905=ADVANCED_FACE ( 'NONE', ( #99268 ), #82528, .T. ) ;
#67906=EDGE_LOOP ( 'NONE', ( #14306, #24949, #17413, #37296 ) ) ;
#67907=AXIS2_PLACEMENT_3D ( 'NONE', #28752, #120354, #1847 ) ;
#67908=ORIENTED_EDGE ( 'NONE', *, *, #83749, .F. ) ;
#67909=ORIENTED_EDGE ( 'NONE', *, *, #32600, .T. ) ;
#67910=EDGE_LOOP ( 'NONE', ( #45819, #116471, #24775, #101683 ) ) ;
#67911=DIRECTION ( 'NONE',  ( -0.000000000000000000, 1.000000000000000000, -0.000000000000000000 ) ) ;
#67912=CARTESIAN_POINT ( 'NONE',  ( 26.76176526818647972, 1.073658814953058815, 4.445806700279154811 ) ) ;
#67913=CONICAL_SURFACE ( 'NONE', #42821, 0.1000000000000002554, 0.003490658503988666988 ) ;
#67914=FACE_OUTER_BOUND ( 'NONE', #56379, .T. ) ;
#67915=FACE_BOUND ( 'NONE', #35488, .T. ) ;
#67916=DIRECTION ( 'NONE',  ( -4.274815082592931898E-19, -0.9999939076577903929, -0.003490651415223739937 ) ) ;
#67918=FACE_OUTER_BOUND ( 'NONE', #54282, .T. ) ;
#67919=LINE ( 'NONE', #37820, #64676 ) ;
#67920=AXIS2_PLACEMENT_3D ( 'NONE', #6315, #75089, #35808 ) ;
#67921=CIRCLE ( 'NONE', #103439, 0.06509327318403745899 ) ;
#67922=AXIS2_PLACEMENT_3D ( 'NONE', #38241, #127265, #67675 ) ;
#67924=DIRECTION ( 'NONE',  ( 0.000000000000000000, 0.000000000000000000, 1.000000000000000000 ) ) ;
#67925=CARTESIAN_POINT ( 'NONE',  ( -2.900000000000029221, 2.500000000000000000, -0.6928203230275541413 ) ) ;
#67926=VECTOR ( 'NONE', #48883, 1000.000000000000000 ) ;
#67927=AXIS2_PLACEMENT_3D ( 'NONE', #104962, #105637, #15291 ) ;
#67928=CARTESIAN_POINT ( 'NONE',  ( -5.000000000000023093, 12.50000000000000000, 0.6928203230275494784 ) ) ;
#67929=ORIENTED_EDGE ( 'NONE', *, *, #82226, .F. ) ;
#67930=ORIENTED_EDGE ( 'NONE', *, *, #63600, .T. ) ;
#67931=ORIENTED_EDGE ( 'NONE', *, *, #110324, .F. ) ;
#67932=ORIENTED_EDGE ( 'NONE', *, *, #45561, .F. ) ;
#67933=VECTOR ( 'NONE', #12157, 1000.000000000000000 ) ;
#67934=DIRECTION ( 'NONE',  ( 0.000000000000000000, 0.000000000000000000, 1.000000000000000000 ) ) ;
#67935=FACE_BOUND ( 'NONE', #46479, .T. ) ;
#67936=DIRECTION ( 'NONE',  ( -4.274815082592931898E-19, -0.9999939076577903929, -0.003490651415223739937 ) ) ;
#67937=ADVANCED_FACE ( 'NONE', ( #86185 ), #7636, .T. ) ;
#67938=ORIENTED_EDGE ( 'NONE', *, *, #87929, .T. ) ;
#67939=FACE_OUTER_BOUND ( 'NONE', #95648, .T. ) ;
#67940=CARTESIAN_POINT ( 'NONE',  ( 12.29999999999990479, 2.500000000000000000, 4.676537180435972552 ) ) ;
#67941=DIRECTION ( 'NONE',  ( 0.000000000000000000, -0.000000000000000000, 1.000000000000000000 ) ) ;
#67942=AXIS2_PLACEMENT_3D ( 'NONE', #70855, #10614, #69553 ) ;
#67943=ORIENTED_EDGE ( 'NONE', *, *, #25325, .F. ) ;
#67945=DIRECTION ( 'NONE',  ( 0.000000000000000000, -0.9999939076577903929, 0.003490651415223739937 ) ) ;
#67946=ADVANCED_FACE ( 'NONE', ( #37123 ), #32373, .T. ) ;
#67948=ORIENTED_EDGE ( 'NONE', *, *, #83399, .T. ) ;
#67949=DIRECTION ( 'NONE',  ( 0.000000000000000000, 0.000000000000000000, 1.000000000000000000 ) ) ;
#67950=FACE_OUTER_BOUND ( 'NONE', #20467, .T. ) ;
#67951=AXIS2_PLACEMENT_3D ( 'NONE', #112885, #62510, #103715 ) ;
#67952=CIRCLE ( 'NONE', #38752, 0.1000000000000002554 ) ;
#67953=DIRECTION ( 'NONE',  ( 0.000000000000000000, 1.000000000000000000, 0.000000000000000000 ) ) ;
#67954=FACE_OUTER_BOUND ( 'NONE', #105976, .T. ) ;
#67955=EDGE_LOOP ( 'NONE', ( #41195, #62515 ) ) ;
#67956=DIRECTION ( 'NONE',  ( 0.000000000000000000, 1.000000000000000000, 0.000000000000000000 ) ) ;
#67957=VERTEX_POINT ( 'NONE', #97322 ) ;
#67958=VERTEX_POINT ( 'NONE', #101835 ) ;
#67959=DIRECTION ( 'NONE',  ( 0.000000000000000000, 1.000000000000000000, 0.000000000000000000 ) ) ;
#67960=EDGE_LOOP ( 'NONE', ( #120187, #15684, #25491, #73988 ) ) ;
#67961=DIRECTION ( 'NONE',  ( 0.000000000000000000, 0.000000000000000000, 1.000000000000000000 ) ) ;
#67962=FACE_BOUND ( 'NONE', #101614, .T. ) ;
#67963=EDGE_LOOP ( 'NONE', ( #90005, #118524 ) ) ;
#67965=ORIENTED_EDGE ( 'NONE', *, *, #15132, .T. ) ;
#67966=DIRECTION ( 'NONE',  ( -0.000000000000000000, 1.000000000000000000, -0.000000000000000000 ) ) ;
#67967=CARTESIAN_POINT ( 'NONE',  ( 10.84999999999991260, 2.500000000000000000, 6.495190528383297135 ) ) ;
#67968=DIRECTION ( 'NONE',  ( -0.000000000000000000, -1.000000000000000000, -0.000000000000000000 ) ) ;
#67969=CARTESIAN_POINT ( 'NONE',  ( 0.8499999999999553468, 2.500000000000000000, -2.857883832488653741 ) ) ;
#67970=PLANE ( 'NONE',  #70435 ) ;
#67971=ORIENTED_EDGE ( 'NONE', *, *, #100537, .F. ) ;
#67972=EDGE_LOOP ( 'NONE', ( #110188, #99078, #38309, #124812 ) ) ;
#67973=EDGE_CURVE ( 'NONE', #128034, #70146, #49083, .T. ) ;
#67974=ORIENTED_EDGE ( 'NONE', *, *, #44800, .F. ) ;
#67975=CARTESIAN_POINT ( 'NONE',  ( -6.250000000000017764, 2.500000000000000000, 7.288010851410849256 ) ) ;
#67976=VECTOR ( 'NONE', #108332, 1000.000000000000000 ) ;
#67977=AXIS2_PLACEMENT_3D ( 'NONE', #59120, #67623, #68923 ) ;
#67978=DIRECTION ( 'NONE',  ( 0.000000000000000000, 0.000000000000000000, -1.000000000000000000 ) ) ;
#67979=DIRECTION ( 'NONE',  ( 0.000000000000000000, -0.000000000000000000, 1.000000000000000000 ) ) ;
#67980=VERTEX_POINT ( 'NONE', #71082 ) ;
#67981=ORIENTED_EDGE ( 'NONE', *, *, #125950, .F. ) ;
#67982=ORIENTED_EDGE ( 'NONE', *, *, #27899, .T. ) ;
#67983=DIRECTION ( 'NONE',  ( 0.000000000000000000, -0.000000000000000000, 1.000000000000000000 ) ) ;
#67984=DIRECTION ( 'NONE',  ( -4.274815082592931898E-19, -0.9999939076577903929, -0.003490651415223739937 ) ) ;
#67985=EDGE_CURVE ( 'NONE', #115300, #129059, #90062, .T. ) ;
#67987=DIRECTION ( 'NONE',  ( 0.000000000000000000, 0.000000000000000000, 1.000000000000000000 ) ) ;
#67988=DIRECTION ( 'NONE',  ( 0.000000000000000000, 0.000000000000000000, 1.000000000000000000 ) ) ;
#67989=AXIS2_PLACEMENT_3D ( 'NONE', #4360, #5019, #124162 ) ;
#67990=CARTESIAN_POINT ( 'NONE',  ( 2.699999999999945555, 12.50000000000000000, 3.918623584224382839 ) ) ;
#67991=CARTESIAN_POINT ( 'NONE',  ( 8.549999999999918998, 12.50000000000000000, -1.818653347947326138 ) ) ;
#67992=CARTESIAN_POINT ( 'NONE',  ( -12.69999999999999396, 2.500000000000000000, -3.983716857408423628 ) ) ;
#67993=EDGE_CURVE ( 'NONE', #101949, #356, #61273, .T. ) ;
#67994=EDGE_CURVE ( 'NONE', #30373, #55743, #69794, .T. ) ;
#67995=AXIS2_PLACEMENT_3D ( 'NONE', #34702, #115808, #64771 ) ;
#67996=CARTESIAN_POINT ( 'NONE',  ( 15.59999999999988951, 2.500000000000000000, -0.4464101615137783252 ) ) ;
#67997=VERTEX_POINT ( 'NONE', #50805 ) ;
#67998=ORIENTED_EDGE ( 'NONE', *, *, #126846, .T. ) ;
#67999=DIRECTION ( 'NONE',  ( -4.274815082592931898E-19, -0.9999939076577903929, -0.003490651415223739937 ) ) ;
#68000=CIRCLE ( 'NONE', #126502, 0.06509327318403745899 ) ;
#68001=EDGE_CURVE ( 'NONE', #48532, #67328, #88960, .T. ) ;
#68002=AXIS2_PLACEMENT_3D ( 'NONE', #84776, #85414, #64483 ) ;
#68003=FACE_OUTER_BOUND ( 'NONE', #113600, .T. ) ;
#68005=ORIENTED_EDGE ( 'NONE', *, *, #10699, .F. ) ;
#68006=VERTEX_POINT ( 'NONE', #72391 ) ;
#68007=ADVANCED_FACE ( 'NONE', ( #2319 ), #30399, .T. ) ;
#68009=CARTESIAN_POINT ( 'NONE',  ( -6.081641213347104214E-15, 12.50000000000000000, -4.395220292106239768 ) ) ;
#68010=DIRECTION ( 'NONE',  ( 0.000000000000000000, 0.000000000000000000, -1.000000000000000000 ) ) ;
#68011=CIRCLE ( 'NONE', #59724, 0.06509327318403745899 ) ;
#68012=FACE_OUTER_BOUND ( 'NONE', #27687, .T. ) ;
#68013=CONICAL_SURFACE ( 'NONE', #128691, 0.1000000000000002554, 0.003490658503988666988 ) ;
#68014=CONICAL_SURFACE ( 'NONE', #86790, 0.1000000000000002554, 0.003490658503988666988 ) ;
#68015=FACE_OUTER_BOUND ( 'NONE', #98514, .T. ) ;
#68016=DIRECTION ( 'NONE',  ( 0.000000000000000000, 0.000000000000000000, 1.000000000000000000 ) ) ;
#68017=DIRECTION ( 'NONE',  ( 0.000000000000000000, 0.000000000000000000, 1.000000000000000000 ) ) ;
#68018=ORIENTED_EDGE ( 'NONE', *, *, #66742, .T. ) ;
#68019=CARTESIAN_POINT ( 'NONE',  ( -8.550000000000013145, 2.500000000000000000, 2.411473670974873862 ) ) ;
#68020=CARTESIAN_POINT ( 'NONE',  ( 3.749999999999978684, 2.500000000000000000, -2.065063509461102065 ) ) ;
#68021=CIRCLE ( 'NONE', #103536, 0.06509327318403745899 ) ;
#68023=ORIENTED_EDGE ( 'NONE', *, *, #40367, .T. ) ;
#68024=VECTOR ( 'NONE', #30991, 1000.000000000000000 ) ;
#68025=ORIENTED_EDGE ( 'NONE', *, *, #109262, .T. ) ;
#68026=EDGE_LOOP ( 'NONE', ( #77839, #59922, #79933, #116077 ) ) ;
#68027=ORIENTED_EDGE ( 'NONE', *, *, #101293, .T. ) ;
#68028=CARTESIAN_POINT ( 'NONE',  ( 11.24999999999990763, 2.500000000000000000, 1.472243186433545459 ) ) ;
#68029=LINE ( 'NONE', #39883, #75112 ) ;
#68030=ORIENTED_EDGE ( 'NONE', *, *, #43262, .F. ) ;
#68031=CARTESIAN_POINT ( 'NONE',  ( 11.64999999999990798, 2.500000000000000000, -1.472243186433550122 ) ) ;
#68032=EDGE_CURVE ( 'NONE', #99852, #35495, #11584, .T. ) ;
#68033=CARTESIAN_POINT ( 'NONE',  ( 6.249999999999965361, 2.500000000000000000, 2.065063509461097624 ) ) ;
#68034=DIRECTION ( 'NONE',  ( 0.000000000000000000, 1.000000000000000000, 0.000000000000000000 ) ) ;
#68035=DIRECTION ( 'NONE',  ( 0.000000000000000000, 0.000000000000000000, -1.000000000000000000 ) ) ;
#68036=ORIENTED_EDGE ( 'NONE', *, *, #704, .F. ) ;
#68037=DIRECTION ( 'NONE',  ( -0.000000000000000000, 1.000000000000000000, -0.000000000000000000 ) ) ;
#68038=CIRCLE ( 'NONE', #111972, 0.1000000000000002554 ) ;
#68039=ADVANCED_FACE ( 'NONE', ( #121457 ), #76350, .T. ) ;
#68040=FACE_OUTER_BOUND ( 'NONE', #129189, .T. ) ;
#68041=VERTEX_POINT ( 'NONE', #110358 ) ;
#68042=EDGE_LOOP ( 'NONE', ( #23158, #104257 ) ) ;
#68043=ORIENTED_EDGE ( 'NONE', *, *, #128758, .F. ) ;
#68044=CARTESIAN_POINT ( 'NONE',  ( 7.699999999999925571, 2.500000000000000000, -4.676537180435978769 ) ) ;
#68045=ADVANCED_FACE ( 'NONE', ( #51461 ), #51324, .T. ) ;
#68046=ADVANCED_FACE ( 'NONE', ( #12148 ), #42277, .T. ) ;
#68047=CIRCLE ( 'NONE', #11615, 0.06509327318403745899 ) ;
#68048=EDGE_CURVE ( 'NONE', #26341, #31641, #31813, .T. ) ;
#68049=CARTESIAN_POINT ( 'NONE',  ( -10.00000000000000533, 2.500000000000000000, 0.7928203230275495672 ) ) ;
#68050=AXIS2_PLACEMENT_3D ( 'NONE', #120107, #48794, #108966 ) ;
#68051=ADVANCED_FACE ( 'NONE', ( #82198 ), #40866, .T. ) ;
#68052=ORIENTED_EDGE ( 'NONE', *, *, #99226, .F. ) ;
#68053=LINE ( 'NONE', #107979, #49527 ) ;
#68054=CARTESIAN_POINT ( 'NONE',  ( 8.349999999999919709, 12.50000000000000000, 5.867463478539781896 ) ) ;
#68055=DIRECTION ( 'NONE',  ( 0.000000000000000000, 1.000000000000000000, 0.000000000000000000 ) ) ;
#68056=CARTESIAN_POINT ( 'NONE',  ( 9.399999999999918643, 12.50000000000000000, -0.4115034346978156399 ) ) ;
#68057=EDGE_CURVE ( 'NONE', #129352, #25026, #113999, .T. ) ;
#68058=VERTEX_POINT ( 'NONE', #99906 ) ;
#68059=ADVANCED_FACE ( 'NONE', ( #22006 ), #34601, .T. ) ;
#68061=CONICAL_SURFACE ( 'NONE', #78554, 0.1000000000000002554, 0.003490658503988666988 ) ;
#68062=VERTEX_POINT ( 'NONE', #62570 ) ;
#68063=ORIENTED_EDGE ( 'NONE', *, *, #120671, .F. ) ;
#68064=CARTESIAN_POINT ( 'NONE',  ( -10.00000000000000355, 12.50000000000000000, -0.6277270498435166823 ) ) ;
#68065=DIRECTION ( 'NONE',  ( 0.000000000000000000, 1.000000000000000000, 0.000000000000000000 ) ) ;
#68066=FACE_BOUND ( 'NONE', #28823, .T. ) ;
#68067=CARTESIAN_POINT ( 'NONE',  ( -10.65000000000000213, 2.500000000000000000, 6.941600689897073018 ) ) ;
#68068=CARTESIAN_POINT ( 'NONE',  ( 0.5999999999999560130, 12.50000000000000000, -4.048810130592463530 ) ) ;
#68070=CIRCLE ( 'NONE', #72296, 0.06509327318403745899 ) ;
#68071=VECTOR ( 'NONE', #121896, 1000.000000000000000 ) ;
#68072=ORIENTED_EDGE ( 'NONE', *, *, #69034, .F. ) ;
#68073=CARTESIAN_POINT ( 'NONE',  ( 1.899999999999951283, 2.500000000000000000, -4.776537180435977525 ) ) ;
#68074=CARTESIAN_POINT ( 'NONE',  ( 10.84999999999990905, 2.500000000000000000, -7.088010851410853519 ) ) ;
#68075=CARTESIAN_POINT ( 'NONE',  ( -0.4500000000000402012, 2.500000000000000000, 2.165063509461097713 ) ) ;
#68077=ORIENTED_EDGE ( 'NONE', *, *, #31590, .T. ) ;
#68078=DIRECTION ( 'NONE',  ( 0.000000000000000000, 1.000000000000000000, 0.000000000000000000 ) ) ;
#68079=FACE_OUTER_BOUND ( 'NONE', #9251, .T. ) ;
#68080=ORIENTED_EDGE ( 'NONE', *, *, #3599, .T. ) ;
#68081=VERTEX_POINT ( 'NONE', #9587 ) ;
#68082=DIRECTION ( 'NONE',  ( 0.000000000000000000, 0.000000000000000000, 1.000000000000000000 ) ) ;
#68083=PLANE ( 'NONE',  #425 ) ;
#68084=FACE_BOUND ( 'NONE', #86327, .T. ) ;
#68085=DIRECTION ( 'NONE',  ( 0.000000000000000000, 1.000000000000000000, 0.000000000000000000 ) ) ;
#68086=AXIS2_PLACEMENT_3D ( 'NONE', #121261, #11298, #110154 ) ;
#68087=VERTEX_POINT ( 'NONE', #109725 ) ;
#68088=CARTESIAN_POINT ( 'NONE',  ( -1.850000000000033396, 2.500000000000000000, -1.718653347947325827 ) ) ;
#68089=AXIS2_PLACEMENT_3D ( 'NONE', #124554, #104883, #105555 ) ;
#68090=ORIENTED_EDGE ( 'NONE', *, *, #70911, .T. ) ;
#68091=ORIENTED_EDGE ( 'NONE', *, *, #114881, .F. ) ;
#68092=FACE_OUTER_BOUND ( 'NONE', #61251, .T. ) ;
#68094=ORIENTED_EDGE ( 'NONE', *, *, #83463, .T. ) ;
#68095=FACE_OUTER_BOUND ( 'NONE', #86582, .T. ) ;
#68096=CARTESIAN_POINT ( 'NONE',  ( -8.150000000000009237, 12.50000000000000000, 6.841600689897072485 ) ) ;
#68097=ADVANCED_FACE ( 'NONE', ( #39722 ), #15683, .T. ) ;
#68098=AXIS2_PLACEMENT_3D ( 'NONE', #108294, #51340, #59879 ) ;
#68099=DIRECTION ( 'NONE',  ( -0.000000000000000000, -1.000000000000000000, -0.000000000000000000 ) ) ;
#68100=CARTESIAN_POINT ( 'NONE',  ( 12.69999999999990159, 2.500000000000000000, -3.883716857408426648 ) ) ;
#68101=AXIS2_PLACEMENT_3D ( 'NONE', #59193, #60489, #100395 ) ;
#68102=CONICAL_SURFACE ( 'NONE', #78318, 0.1000000000000002554, 0.003490658503988666988 ) ;
#68103=ORIENTED_EDGE ( 'NONE', *, *, #74468, .F. ) ;
#68104=CONICAL_SURFACE ( 'NONE', #70279, 0.09999999999999999167, 0.003490658503988666988 ) ;
#68105=DIRECTION ( 'NONE',  ( -0.000000000000000000, 1.000000000000000000, -0.000000000000000000 ) ) ;
#68106=LINE ( 'NONE', #106107, #28883 ) ;
#68107=CARTESIAN_POINT ( 'NONE',  ( 8.149999999999923972, 2.500000000000000000, 1.918653347947321564 ) ) ;
#68108=CIRCLE ( 'NONE', #78324, 0.09999999999999982514 ) ;
#68109=CARTESIAN_POINT ( 'NONE',  ( 6.849999999999929479, 2.500000000000000000, -1.918653347947326004 ) ) ;
#68110=ORIENTED_EDGE ( 'NONE', *, *, #123424, .F. ) ;
#68111=DIRECTION ( 'NONE',  ( 0.000000000000000000, 1.000000000000000000, 0.000000000000000000 ) ) ;
#68113=CARTESIAN_POINT ( 'NONE',  ( 16.88398462908685005, 2.500000000000000000, 4.430583899588694585 ) ) ;
#68114=ORIENTED_EDGE ( 'NONE', *, *, #123517, .F. ) ;
#68115=DIRECTION ( 'NONE',  ( 0.000000000000000000, 1.000000000000000000, 0.000000000000000000 ) ) ;
#68117=DIRECTION ( 'NONE',  ( 0.000000000000000000, 0.000000000000000000, -1.000000000000000000 ) ) ;
#68118=CARTESIAN_POINT ( 'NONE',  ( -8.350000000000010303, 2.500000000000000000, 6.595190528383296780 ) ) ;
#68119=EDGE_LOOP ( 'NONE', ( #21716, #125209, #122583, #18746 ) ) ;
#68120=CARTESIAN_POINT ( 'NONE',  ( 10.59999999999990905, 2.500000000000000000, 4.576537180435972019 ) ) ;
#68121=DIRECTION ( 'NONE',  ( 0.000000000000000000, 1.000000000000000000, 0.000000000000000000 ) ) ;
#68122=FACE_OUTER_BOUND ( 'NONE', #53156, .T. ) ;
#68124=DIRECTION ( 'NONE',  ( -4.274815082592931898E-19, -0.9999939076577903929, -0.003490651415223739937 ) ) ;
#68125=CARTESIAN_POINT ( 'NONE',  ( -13.09999999999999076, 12.50000000000000000, 4.676537180435972552 ) ) ;
#68126=VERTEX_POINT ( 'NONE', #80267 ) ;
#68127=ORIENTED_EDGE ( 'NONE', *, *, #66364, .F. ) ;
#68128=PLANE ( 'NONE',  #116355 ) ;
#68130=DIRECTION ( 'NONE',  ( 0.000000000000000000, -0.9999939076577903929, 0.003490651415223739937 ) ) ;
#68131=ORIENTED_EDGE ( 'NONE', *, *, #62762, .T. ) ;
#68132=EDGE_LOOP ( 'NONE', ( #85354, #113545 ) ) ;
#68133=AXIS2_PLACEMENT_3D ( 'NONE', #73273, #54916, #3254 ) ;
#68134=ORIENTED_EDGE ( 'NONE', *, *, #43972, .F. ) ;
#68135=DIRECTION ( 'NONE',  ( 0.000000000000000000, 0.000000000000000000, 1.000000000000000000 ) ) ;
#68136=VECTOR ( 'NONE', #122523, 1000.000000000000000 ) ;
#68137=CIRCLE ( 'NONE', #11708, 0.06509327318403745899 ) ;
#68138=DIRECTION ( 'NONE',  ( -0.000000000000000000, 1.000000000000000000, -0.000000000000000000 ) ) ;
#68139=EDGE_CURVE ( 'NONE', #115197, #114185, #120266, .T. ) ;
#68140=CARTESIAN_POINT ( 'NONE',  ( -13.09999999999999076, 2.500000000000000000, 3.883716857408421319 ) ) ;
#68141=AXIS2_PLACEMENT_3D ( 'NONE', #29467, #119773, #71308 ) ;
#68142=DIRECTION ( 'NONE',  ( 0.000000000000000000, 0.000000000000000000, -1.000000000000000000 ) ) ;
#68143=LINE ( 'NONE', #99564, #73134 ) ;
#68144=DIRECTION ( 'NONE',  ( 0.000000000000000000, 0.000000000000000000, 1.000000000000000000 ) ) ;
#68145=PLANE ( 'NONE',  #42432 ) ;
#68146=EDGE_CURVE ( 'NONE', #83529, #23572, #38815, .T. ) ;
#68147=EDGE_CURVE ( 'NONE', #115955, #74459, #101484, .T. ) ;
#68148=FACE_OUTER_BOUND ( 'NONE', #97190, .T. ) ;
#68149=ORIENTED_EDGE ( 'NONE', *, *, #34383, .T. ) ;
#68150=AXIS2_PLACEMENT_3D ( 'NONE', #47006, #47646, #37188 ) ;
#68151=ORIENTED_EDGE ( 'NONE', *, *, #18915, .T. ) ;
#68152=ORIENTED_EDGE ( 'NONE', *, *, #39967, .T. ) ;
#68153=VECTOR ( 'NONE', #42573, 1000.000000000000000 ) ;
#68154=AXIS2_PLACEMENT_3D ( 'NONE', #112730, #72804, #42720 ) ;
#68155=EDGE_CURVE ( 'NONE', #10727, #12562, #32464, .T. ) ;
#68156=FACE_OUTER_BOUND ( 'NONE', #110532, .T. ) ;
#68157=ADVANCED_FACE ( 'NONE', ( #75581 ), #105598, .T. ) ;
#68158=EDGE_CURVE ( 'NONE', #86861, #101388, #19919, .T. ) ;
#68159=EDGE_LOOP ( 'NONE', ( #102194, #35022, #77798, #119520 ) ) ;
#68160=ORIENTED_EDGE ( 'NONE', *, *, #128961, .T. ) ;
#68161=EDGE_CURVE ( 'NONE', #6400, #38652, #68021, .T. ) ;
#68162=DIRECTION ( 'NONE',  ( 0.000000000000000000, 1.000000000000000000, 0.000000000000000000 ) ) ;
#68163=DIRECTION ( 'NONE',  ( -4.274815082592931898E-19, -0.9999939076577903929, -0.003490651415223739937 ) ) ;
#68164=DIRECTION ( 'NONE',  ( 0.000000000000000000, 0.000000000000000000, -1.000000000000000000 ) ) ;
#68165=DIRECTION ( 'NONE',  ( 0.000000000000000000, 0.000000000000000000, 1.000000000000000000 ) ) ;
#68166=CARTESIAN_POINT ( 'NONE',  ( 1.649999999999951950, 2.500000000000000000, -7.188010851410854052 ) ) ;
#68167=ORIENTED_EDGE ( 'NONE', *, *, #10129, .F. ) ;
#68168=CARTESIAN_POINT ( 'NONE',  ( -7.100000000000014744, 12.50000000000000000, 4.330127018922196314 ) ) ;
#68169=EDGE_LOOP ( 'NONE', ( #116841, #28134, #122762, #125414 ) ) ;
#68170=CARTESIAN_POINT ( 'NONE',  ( 12.89999999999990088, 2.500000000000000000, -4.230127018922201998 ) ) ;
#68171=ORIENTED_EDGE ( 'NONE', *, *, #104429, .T. ) ;
#68172=DIRECTION ( 'NONE',  ( -0.000000000000000000, -1.000000000000000000, -0.000000000000000000 ) ) ;
#68173=ORIENTED_EDGE ( 'NONE', *, *, #79429, .T. ) ;
#68174=ORIENTED_EDGE ( 'NONE', *, *, #86649, .T. ) ;
#68175=CARTESIAN_POINT ( 'NONE',  ( -15.19999999999998153, 2.500000000000000000, -0.4464101615137759382 ) ) ;
#68176=DIRECTION ( 'NONE',  ( 0.000000000000000000, 0.000000000000000000, 1.000000000000000000 ) ) ;
#68177=CONICAL_SURFACE ( 'NONE', #126683, 0.1000000000000002554, 0.003490658503988666988 ) ;
#68178=FACE_OUTER_BOUND ( 'NONE', #32880, .T. ) ;
#68179=AXIS2_PLACEMENT_3D ( 'NONE', #10548, #50489, #90396 ) ;
#68180=DIRECTION ( 'NONE',  ( -0.000000000000000000, -1.000000000000000000, -0.000000000000000000 ) ) ;
#68181=DIRECTION ( 'NONE',  ( 0.000000000000000000, -0.000000000000000000, 1.000000000000000000 ) ) ;
#68182=ORIENTED_EDGE ( 'NONE', *, *, #114864, .T. ) ;
#68183=DIRECTION ( 'NONE',  ( -4.274815082592931898E-19, -0.9999939076577903929, -0.003490651415223739937 ) ) ;
#68185=ADVANCED_FACE ( 'NONE', ( #74314 ), #114234, .T. ) ;
#68186=DIRECTION ( 'NONE',  ( -4.274815082592931898E-19, -0.9999939076577903929, -0.003490651415223739937 ) ) ;
#68187=DIRECTION ( 'NONE',  ( 0.000000000000000000, -0.9999939076577903929, 0.003490651415223739937 ) ) ;
#68188=CIRCLE ( 'NONE', #20372, 0.06509327318403745899 ) ;
#68189=CIRCLE ( 'NONE', #20087, 0.06509327318403745899 ) ;
#68190=CARTESIAN_POINT ( 'NONE',  ( 5.399999999999934630, 2.500000000000000000, 0.7928203230275495672 ) ) ;
#68191=ORIENTED_EDGE ( 'NONE', *, *, #23892, .F. ) ;
#68192=ORIENTED_EDGE ( 'NONE', *, *, #87597, .F. ) ;
#68193=EDGE_CURVE ( 'NONE', #102955, #118684, #109796, .T. ) ;
#68194=DIRECTION ( 'NONE',  ( 0.000000000000000000, 0.000000000000000000, -1.000000000000000000 ) ) ;
#68195=EDGE_CURVE ( 'NONE', #34456, #40951, #5312, .T. ) ;
#68196=EDGE_CURVE ( 'NONE', #62111, #46500, #45057, .T. ) ;
#68197=ORIENTED_EDGE ( 'NONE', *, *, #54661, .T. ) ;
#68198=CIRCLE ( 'NONE', #118377, 0.06509327318403745899 ) ;
#68199=FACE_OUTER_BOUND ( 'NONE', #58994, .T. ) ;
#68200=CARTESIAN_POINT ( 'NONE',  ( 4.199999999999941558, 2.500000000000000000, -4.330127018922201643 ) ) ;
#68201=AXIS2_PLACEMENT_3D ( 'NONE', #56865, #18248, #105349 ) ;
#68202=EDGE_CURVE ( 'NONE', #74641, #17512, #3197, .T. ) ;
#68203=ORIENTED_EDGE ( 'NONE', *, *, #56485, .T. ) ;
#68205=CARTESIAN_POINT ( 'NONE',  ( -10.20000000000000284, 12.50000000000000000, -0.4115034346978156399 ) ) ;
#68207=DIRECTION ( 'NONE',  ( -4.274815082592931898E-19, -0.9999939076577903929, -0.003490651415223739937 ) ) ;
#68208=CARTESIAN_POINT ( 'NONE',  ( -14.14999999999998614, 12.50000000000000000, -2.099970236277062252 ) ) ;
#68209=ORIENTED_EDGE ( 'NONE', *, *, #4075, .F. ) ;
#68210=EDGE_CURVE ( 'NONE', #101786, #49149, #82613, .T. ) ;
#68211=EDGE_CURVE ( 'NONE', #129348, #35861, #99335, .T. ) ;
#68212=EDGE_CURVE ( 'NONE', #114052, #37015, #36656, .T. ) ;
#68213=CARTESIAN_POINT ( 'NONE',  ( 4.799999999999937650, 12.50000000000000000, -3.983716857408426293 ) ) ;
#68215=PLANE ( 'NONE',  #96596 ) ;
#68216=AXIS2_PLACEMENT_3D ( 'NONE', #103232, #41751, #121564 ) ;
#68217=DIRECTION ( 'NONE',  ( 0.000000000000000000, -0.9999939076577903929, 0.003490651415223739937 ) ) ;
#68218=ADVANCED_FACE ( 'NONE', ( #54647 ), #114861, .T. ) ;
#68219=FACE_OUTER_BOUND ( 'NONE', #61270, .T. ) ;
#68220=EDGE_LOOP ( 'NONE', ( #96790, #91935 ) ) ;
#68221=CIRCLE ( 'NONE', #55702, 0.06509327318403745899 ) ;
#68223=LINE ( 'NONE', #25722, #67729 ) ;
#68224=AXIS2_PLACEMENT_3D ( 'NONE', #77769, #128188, #107887 ) ;
#68225=VERTEX_POINT ( 'NONE', #23256 ) ;
#68226=LINE ( 'NONE', #9313, #62597 ) ;
#68227=CARTESIAN_POINT ( 'NONE',  ( -3.550000000000027356, 2.500000000000000000, -2.511473670974877948 ) ) ;
#68228=AXIS2_PLACEMENT_3D ( 'NONE', #114620, #24959, #125716 ) ;
#68229=DIRECTION ( 'NONE',  ( 0.000000000000000000, 0.000000000000000000, 1.000000000000000000 ) ) ;
#68230=VECTOR ( 'NONE', #102244, 1000.000000000000000 ) ;
#68231=ORIENTED_EDGE ( 'NONE', *, *, #1378, .T. ) ;
#68232=FACE_OUTER_BOUND ( 'NONE', #17112, .T. ) ;
#68233=CIRCLE ( 'NONE', #78726, 0.09999999999999982514 ) ;
#68234=CARTESIAN_POINT ( 'NONE',  ( 11.24999999999994493, 12.50000000000000000, -2.165063509461101710 ) ) ;
#68235=ORIENTED_EDGE ( 'NONE', *, *, #37426, .F. ) ;
#68236=DIRECTION ( 'NONE',  ( -4.274815082592931898E-19, -0.9999939076577903929, -0.003490651415223739937 ) ) ;
#68237=ORIENTED_EDGE ( 'NONE', *, *, #54295, .T. ) ;
#68238=DIRECTION ( 'NONE',  ( 0.000000000000000000, 0.000000000000000000, -1.000000000000000000 ) ) ;
#68239=CIRCLE ( 'NONE', #18064, 0.1000000000000002554 ) ;
#68240=CIRCLE ( 'NONE', #126754, 0.1000000000000002554 ) ;
#68241=AXIS2_PLACEMENT_3D ( 'NONE', #74729, #45278, #77303 ) ;
#68242=VERTEX_POINT ( 'NONE', #63847 ) ;
#68243=FACE_OUTER_BOUND ( 'NONE', #31809, .T. ) ;
#68244=DIRECTION ( 'NONE',  ( 0.000000000000000000, 1.000000000000000000, 0.000000000000000000 ) ) ;
#68245=ORIENTED_EDGE ( 'NONE', *, *, #22119, .F. ) ;
#68246=EDGE_LOOP ( 'NONE', ( #33232, #31552 ) ) ;
#68247=DIRECTION ( 'NONE',  ( 0.000000000000000000, 0.000000000000000000, 1.000000000000000000 ) ) ;
#68248=DIRECTION ( 'NONE',  ( 0.000000000000000000, 0.000000000000000000, -1.000000000000000000 ) ) ;
#68249=EDGE_LOOP ( 'NONE', ( #109348, #64960, #18649, #30612 ) ) ;
#68250=FACE_OUTER_BOUND ( 'NONE', #93327, .T. ) ;
#68251=CARTESIAN_POINT ( 'NONE',  ( -9.350000000000008527, 12.50000000000000000, -6.083687093685483660 ) ) ;
#68252=EDGE_CURVE ( 'NONE', #121281, #38892, #82857, .T. ) ;
#68254=CARTESIAN_POINT ( 'NONE',  ( 3.549999999999941203, 2.500000000000000000, 6.248780366869521430 ) ) ;
#68255=CARTESIAN_POINT ( 'NONE',  ( -1.900000000000034994, 2.500000000000000000, -4.576537180435978236 ) ) ;
#68256=DIRECTION ( 'NONE',  ( 0.000000000000000000, 0.000000000000000000, 1.000000000000000000 ) ) ;
#68257=ORIENTED_EDGE ( 'NONE', *, *, #124497, .T. ) ;
#68259=ORIENTED_EDGE ( 'NONE', *, *, #12348, .T. ) ;
#68260=ORIENTED_EDGE ( 'NONE', *, *, #56749, .T. ) ;
#68261=DIRECTION ( 'NONE',  ( 0.000000000000000000, 1.000000000000000000, 0.000000000000000000 ) ) ;
#68262=CARTESIAN_POINT ( 'NONE',  ( -10.00000000000000533, 2.500000000000000000, 4.922947341949748257 ) ) ;
#68263=DIRECTION ( 'NONE',  ( 0.000000000000000000, 0.000000000000000000, 1.000000000000000000 ) ) ;
#68264=VERTEX_POINT ( 'NONE', #3630 ) ;
#68265=ADVANCED_FACE ( 'NONE', ( #14074 ), #24115, .T. ) ;
#68266=FACE_BOUND ( 'NONE', #94116, .T. ) ;
#68267=ORIENTED_EDGE ( 'NONE', *, *, #49311, .F. ) ;
#68268=DIRECTION ( 'NONE',  ( 0.000000000000000000, 0.000000000000000000, 1.000000000000000000 ) ) ;
#68269=DIRECTION ( 'NONE',  ( -0.000000000000000000, 1.000000000000000000, -0.000000000000000000 ) ) ;
#68270=DIRECTION ( 'NONE',  ( 0.000000000000000000, 0.000000000000000000, 1.000000000000000000 ) ) ;
#68271=AXIS2_PLACEMENT_3D ( 'NONE', #1962, #70713, #42566 ) ;
#68272=CARTESIAN_POINT ( 'NONE',  ( 12.89999999999990266, 12.50000000000000000, 3.637306695894644726 ) ) ;
#68273=CONICAL_SURFACE ( 'NONE', #89213, 0.09999999999999982514, 0.003490658503988666988 ) ;
#68274=DIRECTION ( 'NONE',  ( -4.274815082592931898E-19, -0.9999939076577903929, -0.003490651415223739937 ) ) ;
#68275=DIRECTION ( 'NONE',  ( -0.000000000000000000, -1.000000000000000000, -0.000000000000000000 ) ) ;
#68276=PLANE ( 'NONE',  #49912 ) ;
#68277=FACE_OUTER_BOUND ( 'NONE', #12599, .T. ) ;
#68278=DIRECTION ( 'NONE',  ( -4.274815082592931898E-19, -0.9999939076577903929, -0.003490651415223739937 ) ) ;
#68279=CARTESIAN_POINT ( 'NONE',  ( 3.749999999999978684, 2.500000000000000000, -2.065063509461102065 ) ) ;
#68280=AXIS2_PLACEMENT_3D ( 'NONE', #53091, #104738, #14428 ) ;
#68282=VERTEX_POINT ( 'NONE', #6820 ) ;
#68283=EDGE_LOOP ( 'NONE', ( #33909, #116139 ) ) ;
#68284=EDGE_LOOP ( 'NONE', ( #46399, #65751, #68257, #30006 ) ) ;
#68285=EDGE_LOOP ( 'NONE', ( #20374, #129063 ) ) ;
#68286=FACE_OUTER_BOUND ( 'NONE', #82641, .T. ) ;
#68287=DIRECTION ( 'NONE',  ( 0.000000000000000000, 0.000000000000000000, -1.000000000000000000 ) ) ;
#68288=ORIENTED_EDGE ( 'NONE', *, *, #7478, .T. ) ;
#68289=ORIENTED_EDGE ( 'NONE', *, *, #61082, .T. ) ;
#68290=ORIENTED_EDGE ( 'NONE', *, *, #88566, .F. ) ;
#68291=FACE_OUTER_BOUND ( 'NONE', #100096, .T. ) ;
#68292=AXIS2_PLACEMENT_3D ( 'NONE', #128974, #59592, #28822 ) ;
#68293=CIRCLE ( 'NONE', #116403, 0.1000000000000000472 ) ;
#68294=EDGE_CURVE ( 'NONE', #60265, #73054, #7371, .T. ) ;
#68295=CARTESIAN_POINT ( 'NONE',  ( -4.121192902244064579E-14, 2.500000000000000000, 3.537306695894645081 ) ) ;
#68296=CARTESIAN_POINT ( 'NONE',  ( 1.649999999999948841, 2.500000000000000000, 6.595190528383296780 ) ) ;
#68297=FACE_OUTER_BOUND ( 'NONE', #18617, .T. ) ;
#68298=DIRECTION ( 'NONE',  ( -4.274815082592931898E-19, -0.9999939076577903929, -0.003490651415223739937 ) ) ;
#68299=CARTESIAN_POINT ( 'NONE',  ( -1.050000000000038680, 12.50000000000000000, 6.841600689897072485 ) ) ;
#68300=DIRECTION ( 'NONE',  ( -0.000000000000000000, 1.000000000000000000, -0.000000000000000000 ) ) ;
#68301=ORIENTED_EDGE ( 'NONE', *, *, #66804, .T. ) ;
#68302=EDGE_CURVE ( 'NONE', #123305, #26624, #74374, .T. ) ;
#68303=DIRECTION ( 'NONE',  ( -0.000000000000000000, 1.000000000000000000, -0.000000000000000000 ) ) ;
#68304=ORIENTED_EDGE ( 'NONE', *, *, #34235, .F. ) ;
#68305=ORIENTED_EDGE ( 'NONE', *, *, #31437, .T. ) ;
#68306=VERTEX_POINT ( 'NONE', #17957 ) ;
#68307=ADVANCED_FACE ( 'NONE', ( #36340 ), #105772, .T. ) ;
#68308=DIRECTION ( 'NONE',  ( 0.000000000000000000, -0.9999939076577903929, 0.003490651415223739937 ) ) ;
#68309=ADVANCED_FACE ( 'NONE', ( #76887 ), #118737, .T. ) ;
#68310=EDGE_CURVE ( 'NONE', #48350, #104335, #30490, .T. ) ;
#68311=ORIENTED_EDGE ( 'NONE', *, *, #41031, .F. ) ;
#68312=ADVANCED_FACE ( 'NONE', ( #66410 ), #124561, .T. ) ;
#68313=CIRCLE ( 'NONE', #74579, 0.06509327318403745899 ) ;
#68314=EDGE_CURVE ( 'NONE', #64309, #59989, #97168, .T. ) ;
#68315=EDGE_LOOP ( 'NONE', ( #35986, #98887, #112482, #59805 ) ) ;
#68316=AXIS2_PLACEMENT_3D ( 'NONE', #57678, #4671, #45283 ) ;
#68317=DIRECTION ( 'NONE',  ( 0.000000000000000000, 0.000000000000000000, 1.000000000000000000 ) ) ;
#68318=PLANE ( 'NONE',  #66377 ) ;
#68319=DIRECTION ( 'NONE',  ( -0.000000000000000000, -1.000000000000000000, -0.000000000000000000 ) ) ;
#68320=AXIS2_PLACEMENT_3D ( 'NONE', #21223, #52616, #91260 ) ;
#68321=DIRECTION ( 'NONE',  ( -4.274815082592931898E-19, -0.9999939076577903929, -0.003490651415223739937 ) ) ;
#68322=CARTESIAN_POINT ( 'NONE',  ( -7.050000000000016698, 12.50000000000000000, -6.430097255199264339 ) ) ;
#68323=ADVANCED_FACE ( 'NONE', ( #87330 ), #13722, .T. ) ;
#68324=CIRCLE ( 'NONE', #60034, 0.09999999999999982514 ) ;
#68325=VERTEX_POINT ( 'NONE', #67696 ) ;
#68326=DIRECTION ( 'NONE',  ( -0.000000000000000000, 1.000000000000000000, -0.000000000000000000 ) ) ;
#68327=AXIS2_PLACEMENT_3D ( 'NONE', #80996, #18194, #98050 ) ;
#68329=EDGE_CURVE ( 'NONE', #15286, #111656, #55947, .T. ) ;
#68330=EDGE_LOOP ( 'NONE', ( #125571, #9144 ) ) ;
#68331=CIRCLE ( 'NONE', #83023, 0.1000000000000000056 ) ;
#68332=CARTESIAN_POINT ( 'NONE',  ( -3.150000000000032330, 12.50000000000000000, -6.148780366869526226 ) ) ;
#68333=EDGE_LOOP ( 'NONE', ( #74903, #78133 ) ) ;
#68334=CARTESIAN_POINT ( 'NONE',  ( 1.449999999999952660, 12.50000000000000000, -6.906693963081115939 ) ) ;
#68335=CARTESIAN_POINT ( 'NONE',  ( 3.749999999999942268, 12.50000000000000000, 1.537336459617582918 ) ) ;
#68336=ORIENTED_EDGE ( 'NONE', *, *, #44274, .T. ) ;
#68337=DIRECTION ( 'NONE',  ( 0.000000000000000000, 0.000000000000000000, -1.000000000000000000 ) ) ;
#68338=CONICAL_SURFACE ( 'NONE', #118502, 0.09999999999999982514, 0.003490658503988666988 ) ;
#68339=CARTESIAN_POINT ( 'NONE',  ( 12.09999999999990550, 2.500000000000000000, -4.430127018922202176 ) ) ;
#68340=ORIENTED_EDGE ( 'NONE', *, *, #3345, .T. ) ;
#68341=CIRCLE ( 'NONE', #74605, 0.06509327318403745899 ) ;
#68342=AXIS2_PLACEMENT_3D ( 'NONE', #129363, #28561, #108398 ) ;
#68343=CIRCLE ( 'NONE', #28647, 0.06509327318403745899 ) ;
#68344=PLANE ( 'NONE',  #80175 ) ;
#68345=ORIENTED_EDGE ( 'NONE', *, *, #27666, .F. ) ;
#68346=VERTEX_POINT ( 'NONE', #65763 ) ;
#68347=CARTESIAN_POINT ( 'NONE',  ( 4.599999999999935696, 2.500000000000000000, 5.022947341949748790 ) ) ;
#68348=DIRECTION ( 'NONE',  ( 0.000000000000000000, 0.000000000000000000, -1.000000000000000000 ) ) ;
#68350=LINE ( 'NONE', #30385, #122311 ) ;
#68351=CARTESIAN_POINT ( 'NONE',  ( 2.949999999999946887, 2.500000000000000000, -6.495190528383302464 ) ) ;
#68352=DIRECTION ( 'NONE',  ( 0.000000000000000000, 0.000000000000000000, 1.000000000000000000 ) ) ;
#68353=AXIS2_PLACEMENT_3D ( 'NONE', #125446, #97915, #16111 ) ;
#68354=ORIENTED_EDGE ( 'NONE', *, *, #101548, .F. ) ;
#68355=CARTESIAN_POINT ( 'NONE',  ( 12.94999999999989981, 2.500000000000000000, -2.165063509461101710 ) ) ;
#68356=CARTESIAN_POINT ( 'NONE',  ( -7.500000000000016875, 12.50000000000000000, 0.6277270498435120194 ) ) ;
#68357=VERTEX_POINT ( 'NONE', #78840 ) ;
#68358=CARTESIAN_POINT ( 'NONE',  ( -14.34999999999998543, 2.500000000000000000, 1.818653347947325472 ) ) ;
#68359=CARTESIAN_POINT ( 'NONE',  ( -10.60000000000000320, 2.500000000000000000, -4.676537180435973440 ) ) ;
#68360=DIRECTION ( 'NONE',  ( -0.000000000000000000, 1.000000000000000000, -0.000000000000000000 ) ) ;
#68361=EDGE_CURVE ( 'NONE', #120638, #63670, #91101, .T. ) ;
#68363=CARTESIAN_POINT ( 'NONE',  ( -7.500000000000016875, 2.500000000000000000, 0.7928203230275495672 ) ) ;
#68364=ORIENTED_EDGE ( 'NONE', *, *, #95264, .T. ) ;
#68365=EDGE_CURVE ( 'NONE', #51796, #79506, #36736, .T. ) ;
#68366=AXIS2_PLACEMENT_3D ( 'NONE', #115789, #56216, #96147 ) ;
#68367=AXIS2_PLACEMENT_3D ( 'NONE', #106990, #64025, #56598 ) ;
#68368=EDGE_CURVE ( 'NONE', #67262, #27243, #34692, .T. ) ;
#68369=DIRECTION ( 'NONE',  ( 0.000000000000000000, 0.000000000000000000, -1.000000000000000000 ) ) ;
#68370=LINE ( 'NONE', #36989, #35075 ) ;
#68371=ORIENTED_EDGE ( 'NONE', *, *, #122981, .F. ) ;
#68372=EDGE_CURVE ( 'NONE', #15536, #92369, #6191, .T. ) ;
#68373=AXIS2_PLACEMENT_3D ( 'NONE', #58254, #35383, #107334 ) ;
#68374=AXIS2_PLACEMENT_3D ( 'NONE', #81717, #52276, #3176 ) ;
#68375=CARTESIAN_POINT ( 'NONE',  ( 1.449999999999951328, 12.50000000000000000, -1.818653347947326138 ) ) ;
#68376=ORIENTED_EDGE ( 'NONE', *, *, #66156, .F. ) ;
#68377=VERTEX_POINT ( 'NONE', #116151 ) ;
#68378=DIRECTION ( 'NONE',  ( 0.000000000000000000, 0.000000000000000000, 1.000000000000000000 ) ) ;
#68379=ORIENTED_EDGE ( 'NONE', *, *, #31477, .F. ) ;
#68380=CARTESIAN_POINT ( 'NONE',  ( 12.09999999999990550, 2.500000000000000000, -5.122947341949753763 ) ) ;
#68381=CARTESIAN_POINT ( 'NONE',  ( 4.399999999999939071, 12.50000000000000000, 0.3464101615137736845 ) ) ;
#68382=AXIS2_PLACEMENT_3D ( 'NONE', #98601, #39736, #128093 ) ;
#68383=VECTOR ( 'NONE', #120417, 1000.000000000000000 ) ;
#68384=LINE ( 'NONE', #60369, #112818 ) ;
#68385=ORIENTED_EDGE ( 'NONE', *, *, #98468, .T. ) ;
#68386=CIRCLE ( 'NONE', #76715, 0.1000000000000002554 ) ;
#68387=DIRECTION ( 'NONE',  ( 0.000000000000000000, 0.000000000000000000, -1.000000000000000000 ) ) ;
#68388=CARTESIAN_POINT ( 'NONE',  ( -3.950000000000024603, 2.500000000000000000, 1.818653347947321475 ) ) ;
#68389=VERTEX_POINT ( 'NONE', #26505 ) ;
#68390=FACE_OUTER_BOUND ( 'NONE', #127334, .T. ) ;
#68391=DIRECTION ( 'NONE',  ( 0.000000000000000000, 1.000000000000000000, 0.000000000000000000 ) ) ;
#68392=ADVANCED_FACE ( 'NONE', ( #56578 ), #84831, .T. ) ;
#68393=VERTEX_POINT ( 'NONE', #86702 ) ;
#68394=VERTEX_POINT ( 'NONE', #126637 ) ;
#68395=EDGE_LOOP ( 'NONE', ( #108454, #75842, #122509, #110165 ) ) ;
#68396=LINE ( 'NONE', #57302, #102739 ) ;
#68397=CARTESIAN_POINT ( 'NONE',  ( -4.150000000000028777, 2.500000000000000000, -5.702370205355749455 ) ) ;
#68398=CARTESIAN_POINT ( 'NONE',  ( -3.950000000000026379, 12.50000000000000000, 2.511473670974873507 ) ) ;
#68399=FACE_BOUND ( 'NONE', #45477, .T. ) ;
#68400=ORIENTED_EDGE ( 'NONE', *, *, #24859, .F. ) ;
#68401=DIRECTION ( 'NONE',  ( 0.000000000000000000, 1.000000000000000000, 0.000000000000000000 ) ) ;
#68402=DIRECTION ( 'NONE',  ( 0.000000000000000000, 0.000000000000000000, -1.000000000000000000 ) ) ;
#68403=EDGE_LOOP ( 'NONE', ( #13999, #28920 ) ) ;
#68404=DIRECTION ( 'NONE',  ( 0.000000000000000000, 0.000000000000000000, 1.000000000000000000 ) ) ;
#68405=CARTESIAN_POINT ( 'NONE',  ( 12.49999999999993605, 2.500000000000000000, -0.1000000000000022815 ) ) ;
#68406=AXIS2_PLACEMENT_3D ( 'NONE', #51975, #110237, #20573 ) ;
#68407=EDGE_CURVE ( 'NONE', #75029, #39867, #28417, .T. ) ;
#68408=LINE ( 'NONE', #50094, #98755 ) ;
#68409=DIRECTION ( 'NONE',  ( -0.000000000000000000, 1.000000000000000000, -0.000000000000000000 ) ) ;
#68410=FACE_OUTER_BOUND ( 'NONE', #106763, .T. ) ;
#68411=CARTESIAN_POINT ( 'NONE',  ( 6.049999999999934097, 2.500000000000000000, -2.611473670974877592 ) ) ;
#68412=AXIS2_PLACEMENT_3D ( 'NONE', #62508, #13379, #63788 ) ;
#68413=CARTESIAN_POINT ( 'NONE',  ( 0.8499999999999545697, 2.500000000000000000, 2.757883832488649656 ) ) ;
#68415=CIRCLE ( 'NONE', #37137, 0.09999999999999982514 ) ;
#68416=AXIS2_PLACEMENT_3D ( 'NONE', #100107, #71945, #51662 ) ;
#68417=VERTEX_POINT ( 'NONE', #110217 ) ;
#68418=EDGE_LOOP ( 'NONE', ( #88696, #25262 ) ) ;
#68419=ORIENTED_EDGE ( 'NONE', *, *, #13941, .T. ) ;
#68420=ORIENTED_EDGE ( 'NONE', *, *, #93314, .F. ) ;
#68421=ORIENTED_EDGE ( 'NONE', *, *, #101434, .T. ) ;
#68422=DIRECTION ( 'NONE',  ( 0.000000000000000000, -0.9999939076577903929, 0.003490651415223739937 ) ) ;
#68423=DIRECTION ( 'NONE',  ( 0.000000000000000000, 0.000000000000000000, -1.000000000000000000 ) ) ;
#68424=AXIS2_PLACEMENT_3D ( 'NONE', #128874, #119025, #28069 ) ;
#68425=ORIENTED_EDGE ( 'NONE', *, *, #4776, .F. ) ;
#68427=FACE_BOUND ( 'NONE', #40772, .T. ) ;
#68428=DIRECTION ( 'NONE',  ( -0.000000000000000000, 1.000000000000000000, -0.000000000000000000 ) ) ;
#68429=AXIS2_PLACEMENT_3D ( 'NONE', #108245, #27744, #78811 ) ;
#68430=DIRECTION ( 'NONE',  ( 0.000000000000000000, 0.000000000000000000, -1.000000000000000000 ) ) ;
#68431=DIRECTION ( 'NONE',  ( 0.000000000000000000, 0.000000000000000000, 1.000000000000000000 ) ) ;
#68432=DIRECTION ( 'NONE',  ( -0.000000000000000000, 1.000000000000000000, -0.000000000000000000 ) ) ;
#68433=CARTESIAN_POINT ( 'NONE',  ( 5.849999999999933031, 12.50000000000000000, -1.472243186433550122 ) ) ;
#68434=VERTEX_POINT ( 'NONE', #61108 ) ;
#68435=EDGE_LOOP ( 'NONE', ( #108250, #28311 ) ) ;
#68436=ORIENTED_EDGE ( 'NONE', *, *, #103486, .F. ) ;
#68437=EDGE_LOOP ( 'NONE', ( #53188, #103118 ) ) ;
#68438=DIRECTION ( 'NONE',  ( 0.000000000000000000, -0.9999939076577903929, 0.003490651415223739937 ) ) ;
#68439=DIRECTION ( 'NONE',  ( 0.000000000000000000, 1.000000000000000000, 0.000000000000000000 ) ) ;
#68440=DIRECTION ( 'NONE',  ( -0.000000000000000000, 1.000000000000000000, -0.000000000000000000 ) ) ;
#68441=ORIENTED_EDGE ( 'NONE', *, *, #12365, .T. ) ;
#68442=AXIS2_PLACEMENT_3D ( 'NONE', #69097, #98543, #8882 ) ;
#68443=CARTESIAN_POINT ( 'NONE',  ( 14.79999999999989235, 2.500000000000000000, 0.3464101615137735735 ) ) ;
#68444=DIRECTION ( 'NONE',  ( 0.000000000000000000, -0.9999939076577903929, 0.003490651415223739937 ) ) ;
#68445=EDGE_CURVE ( 'NONE', #119116, #34711, #19909, .T. ) ;
#68446=CARTESIAN_POINT ( 'NONE',  ( -6.900000000000019007, 2.500000000000000000, -3.983716857408426293 ) ) ;
#68448=LINE ( 'NONE', #79577, #115655 ) ;
#68449=CARTESIAN_POINT ( 'NONE',  ( 10.39999999999991154, 12.50000000000000000, -3.637306695894650055 ) ) ;
#68450=DIRECTION ( 'NONE',  ( -4.274815082592931898E-19, -0.9999939076577903929, -0.003490651415223739937 ) ) ;
#68451=ORIENTED_EDGE ( 'NONE', *, *, #49900, .F. ) ;
#68452=CARTESIAN_POINT ( 'NONE',  ( -5.450000000000023270, 12.50000000000000000, -2.165063509461101710 ) ) ;
#68453=ADVANCED_FACE ( 'NONE', ( #40189 ), #82029, .T. ) ;
#68454=CONICAL_SURFACE ( 'NONE', #118629, 0.1000000000000000472, 0.003490658503988666988 ) ;
#68455=ORIENTED_EDGE ( 'NONE', *, *, #125046, .T. ) ;
#68456=VERTEX_POINT ( 'NONE', #899 ) ;
#68457=DIRECTION ( 'NONE',  ( 0.000000000000000000, 1.000000000000000000, 0.000000000000000000 ) ) ;
#68458=EDGE_CURVE ( 'NONE', #55788, #99080, #40958, .T. ) ;
#68459=LINE ( 'NONE', #16764, #67603 ) ;
#68460=FACE_OUTER_BOUND ( 'NONE', #65909, .T. ) ;
#68461=EDGE_CURVE ( 'NONE', #97339, #98598, #38908, .T. ) ;
#68462=ADVANCED_FACE ( 'NONE', ( #80761 ), #80648, .T. ) ;
#68463=EDGE_CURVE ( 'NONE', #84736, #117651, #93174, .T. ) ;
#68464=VERTEX_POINT ( 'NONE', #120681 ) ;
#68465=CIRCLE ( 'NONE', #120704, 0.06509327318403745899 ) ;
#68467=CARTESIAN_POINT ( 'NONE',  ( 8.349999999999919709, 12.50000000000000000, 7.253104124594885960 ) ) ;
#68468=AXIS2_PLACEMENT_3D ( 'NONE', #86498, #74760, #53823 ) ;
#68469=DIRECTION ( 'NONE',  ( -4.274815082592931898E-19, -0.9999939076577903929, -0.003490651415223739937 ) ) ;
#68470=ADVANCED_FACE ( 'NONE', ( #51946 ), #32646, .T. ) ;
#68471=DIRECTION ( 'NONE',  ( -0.000000000000000000, 1.000000000000000000, -0.000000000000000000 ) ) ;
#68472=ORIENTED_EDGE ( 'NONE', *, *, #110712, .T. ) ;
#68473=ORIENTED_EDGE ( 'NONE', *, *, #60957, .F. ) ;
#68474=ADVANCED_FACE ( 'NONE', ( #79478 ), #112035, .T. ) ;
#68475=DIRECTION ( 'NONE',  ( 0.000000000000000000, -0.000000000000000000, 1.000000000000000000 ) ) ;
#68476=EDGE_CURVE ( 'NONE', #51418, #11992, #70932, .T. ) ;
#68477=AXIS2_PLACEMENT_3D ( 'NONE', #9454, #125982, #36354 ) ;
#68478=ORIENTED_EDGE ( 'NONE', *, *, #124814, .F. ) ;
#68479=DIRECTION ( 'NONE',  ( 0.000000000000000000, 1.000000000000000000, 0.000000000000000000 ) ) ;
#68480=EDGE_CURVE ( 'NONE', #28877, #35030, #69639, .T. ) ;
#68481=AXIS2_PLACEMENT_3D ( 'NONE', #62961, #74716, #93083 ) ;
#68482=EDGE_CURVE ( 'NONE', #116451, #103569, #86887, .T. ) ;
#68483=ORIENTED_EDGE ( 'NONE', *, *, #66722, .F. ) ;
#68484=DIRECTION ( 'NONE',  ( 0.000000000000000000, 1.000000000000000000, 0.000000000000000000 ) ) ;
#68485=CARTESIAN_POINT ( 'NONE',  ( -2.900000000000029665, 12.50000000000000000, 3.637306695894644726 ) ) ;
#68487=FACE_OUTER_BOUND ( 'NONE', #62699, .T. ) ;
#68488=ADVANCED_FACE ( 'NONE', ( #2179 ), #32543, .T. ) ;
#68489=VERTEX_POINT ( 'NONE', #129237 ) ;
#68490=DIRECTION ( 'NONE',  ( 0.000000000000000000, 0.000000000000000000, 1.000000000000000000 ) ) ;
#68491=AXIS2_PLACEMENT_3D ( 'NONE', #91951, #71662, #111588 ) ;
#68492=CONICAL_SURFACE ( 'NONE', #5777, 0.1000000000000002554, 0.003490658503988666988 ) ;
#68493=EDGE_LOOP ( 'NONE', ( #1582, #71537, #36614, #84481 ) ) ;
#68494=ORIENTED_EDGE ( 'NONE', *, *, #25060, .T. ) ;
#68495=FACE_OUTER_BOUND ( 'NONE', #55588, .T. ) ;
#68496=PLANE ( 'NONE',  #128509 ) ;
#68497=CARTESIAN_POINT ( 'NONE',  ( -1.050000000000037792, 2.500000000000000000, 6.248780366869520542 ) ) ;
#68499=CIRCLE ( 'NONE', #112523, 0.1000000000000002554 ) ;
#68500=CARTESIAN_POINT ( 'NONE',  ( 0.3999999999999628852, 2.500000000000000000, -0.5928203230275519431 ) ) ;
#68501=AXIS2_PLACEMENT_3D ( 'NONE', #109771, #27985, #17503 ) ;
#68502=CARTESIAN_POINT ( 'NONE',  ( -14.39999999999998614, 2.500000000000000000, 0.4464101615137758272 ) ) ;
#68503=CARTESIAN_POINT ( 'NONE',  ( -0.4000000000000396572, 2.500000000000000000, 3.637306695894644726 ) ) ;
#68504=DIRECTION ( 'NONE',  ( -0.000000000000000000, 1.000000000000000000, -0.000000000000000000 ) ) ;
#68505=CARTESIAN_POINT ( 'NONE',  ( 5.849999999999935696, 2.500000000000000000, -7.188010851410854052 ) ) ;
#68506=CIRCLE ( 'NONE', #85240, 0.09999999999999982514 ) ;
#68507=AXIS2_PLACEMENT_3D ( 'NONE', #101130, #102421, #82795 ) ;
#68508=FACE_OUTER_BOUND ( 'NONE', #31968, .T. ) ;
#68509=CIRCLE ( 'NONE', #85244, 0.06509327318403745899 ) ;
#68510=VERTEX_POINT ( 'NONE', #59854 ) ;
#68511=LINE ( 'NONE', #8297, #42210 ) ;
#68512=LINE ( 'NONE', #49542, #4000 ) ;
#68513=CARTESIAN_POINT ( 'NONE',  ( 0.8499999999999527933, 12.50000000000000000, 7.188010851410848723 ) ) ;
#68514=DIRECTION ( 'NONE',  ( -0.000000000000000000, -1.000000000000000000, -0.000000000000000000 ) ) ;
#68515=CARTESIAN_POINT ( 'NONE',  ( -3.469446951953614189E-14, 2.500000000000000000, -0.6928203230275519209 ) ) ;
#68516=EDGE_LOOP ( 'NONE', ( #1323, #27140, #120428, #102373 ) ) ;
#68517=DIRECTION ( 'NONE',  ( 0.000000000000000000, 1.000000000000000000, 0.000000000000000000 ) ) ;
#68518=EDGE_CURVE ( 'NONE', #68896, #107669, #99112, .T. ) ;
#68519=AXIS2_PLACEMENT_3D ( 'NONE', #34871, #83930, #5375 ) ;
#68520=VECTOR ( 'NONE', #116675, 1000.000000000000000 ) ;
#68521=EDGE_CURVE ( 'NONE', #90590, #60385, #105686, .T. ) ;
#68522=DIRECTION ( 'NONE',  ( -0.000000000000000000, 1.000000000000000000, -0.000000000000000000 ) ) ;
#68523=CARTESIAN_POINT ( 'NONE',  ( 9.999999999999912959, 2.500000000000000000, -5.122947341949753763 ) ) ;
#68524=EDGE_LOOP ( 'NONE', ( #105119, #44161, #129090, #64088 ) ) ;
#68525=( BOUNDED_SURFACE ( )  B_SPLINE_SURFACE ( 3, 2, ( 
 ( #54750, #94683, #45607 ),
 ( #97266, #75056, #75678 ),
 ( #14808, #17396, #124804 ),
 ( #116889, #46890, #96602 ),
 ( #77615, #5008, #44958 ),
 ( #6922, #84867, #114958 ),
 ( #7588, #117520, #107073 ),
 ( #95339, #35150, #27883 ),
 ( #87437, #27231, #105144 ),
 ( #65211, #15473, #95983 ),
 ( #126736, #65871, #85515 ),
 ( #57346, #35775, #55417 ),
 ( #5649, #105803, #115602 ),
 ( #127383, #25959, #6284 ),
 ( #86133, #126072, #36440 ),
 ( #76348, #76986, #47534 ) ),
 .UNSPECIFIED., .F., .F., .F. ) 
 B_SPLINE_SURFACE_WITH_KNOTS ( ( 4, 2, 2, 2, 2, 2, 2, 4 ),
 ( 3, 3 ),
 ( 0.000000000000000000, 0.003502803217043997438, 0.007005606434087994876, 0.008757008042609993811, 0.01050840965113199188, 0.01225981125965399168, 0.01313551206391498985, 0.01401121286817598975 ),
 ( 0.000000000000000000, 1.000000000000000000 ),
 .UNSPECIFIED. ) 
 GEOMETRIC_REPRESENTATION_ITEM ( )  RATIONAL_B_SPLINE_SURFACE ( (
 ( 1.000000000000000000, 0.7071067811865477948, 1.000000000000000000),
 ( 1.000000000000000000, 0.7071067811865477948, 1.000000000000000000),
 ( 1.000000000000000000, 0.7071067811865476838, 1.000000000000000000),
 ( 1.000000000000000000, 0.7071067811865476838, 1.000000000000000000),
 ( 1.000000000000000000, 0.7071067811865476838, 1.000000000000000000),
 ( 1.000000000000000000, 0.7071067811865476838, 1.000000000000000000),
 ( 1.000000000000000000, 0.7071067811865473507, 1.000000000000000000),
 ( 1.000000000000000000, 0.7071067811865473507, 1.000000000000000000),
 ( 1.000000000000000000, 0.7071067811865475727, 1.000000000000000000),
 ( 1.000000000000000000, 0.7071067811865475727, 1.000000000000000000),
 ( 1.000000000000000000, 0.7071067811865477948, 1.000000000000000000),
 ( 1.000000000000000000, 0.7071067811865477948, 1.000000000000000000),
 ( 1.000000000000000000, 0.7071067811865476838, 1.000000000000000000),
 ( 1.000000000000000000, 0.7071067811865476838, 1.000000000000000000),
 ( 1.000000000000000000, 0.7071067811865476838, 1.000000000000000000),
 ( 1.000000000000000000, 0.7071067811865476838, 1.000000000000000000) ) ) 
 REPRESENTATION_ITEM ( '' )  SURFACE ( )  );
#68526=ORIENTED_EDGE ( 'NONE', *, *, #2067, .F. ) ;
#68527=EDGE_CURVE ( 'NONE', #1406, #71123, #103630, .T. ) ;
#68528=CARTESIAN_POINT ( 'NONE',  ( 10.39999999999991154, 2.500000000000000000, 3.637306695894644726 ) ) ;
#68529=ADVANCED_FACE ( 'NONE', ( #242 ), #126620, .T. ) ;
#68530=VERTEX_POINT ( 'NONE', #122615 ) ;
#68531=ORIENTED_EDGE ( 'NONE', *, *, #50913, .F. ) ;
#68532=ORIENTED_EDGE ( 'NONE', *, *, #38811, .T. ) ;
#68533=CARTESIAN_POINT ( 'NONE',  ( 14.34999999999989306, 2.500000000000000000, -2.611473670974877592 ) ) ;
#68534=DIRECTION ( 'NONE',  ( 0.000000000000000000, 0.000000000000000000, 1.000000000000000000 ) ) ;
#68535=CARTESIAN_POINT ( 'NONE',  ( -1.850000000000033396, 12.50000000000000000, -2.511473670974877948 ) ) ;
#68536=CARTESIAN_POINT ( 'NONE',  ( -4.150000000000024336, 12.50000000000000000, -2.857883832488653741 ) ) ;
#68537=ORIENTED_EDGE ( 'NONE', *, *, #99979, .F. ) ;
#68538=CARTESIAN_POINT ( 'NONE',  ( 2.899999999999946620, 12.50000000000000000, 0.6277270498435120194 ) ) ;
#68539=ORIENTED_EDGE ( 'NONE', *, *, #101532, .F. ) ;
#68540=FACE_OUTER_BOUND ( 'NONE', #109165, .T. ) ;
#68541=FACE_OUTER_BOUND ( 'NONE', #68981, .T. ) ;
#68542=AXIS2_PLACEMENT_3D ( 'NONE', #75052, #25281, #45602 ) ;
#68543=CARTESIAN_POINT ( 'NONE',  ( 3.349999999999941025, 2.500000000000000000, 7.188010851410848723 ) ) ;
#68544=CARTESIAN_POINT ( 'NONE',  ( -9.800000000000004263, 12.50000000000000000, -0.3464101615137783474 ) ) ;
#68545=DIRECTION ( 'NONE',  ( 0.000000000000000000, 0.000000000000000000, -1.000000000000000000 ) ) ;
#68546=ORIENTED_EDGE ( 'NONE', *, *, #97544, .T. ) ;
#68547=CONICAL_SURFACE ( 'NONE', #110325, 0.09999999999999982514, 0.003490658503988666988 ) ;
#68548=CIRCLE ( 'NONE', #12116, 0.06509327318403745899 ) ;
#68549=EDGE_LOOP ( 'NONE', ( #23113, #124724, #119326, #122733 ) ) ;
#68550=ORIENTED_EDGE ( 'NONE', *, *, #123170, .F. ) ;
#68551=ORIENTED_EDGE ( 'NONE', *, *, #129499, .F. ) ;
#68552=ORIENTED_EDGE ( 'NONE', *, *, #63070, .T. ) ;
#68553=CARTESIAN_POINT ( 'NONE',  ( 11.84999999999990727, 2.500000000000000000, 6.148780366869520009 ) ) ;
#68554=DIRECTION ( 'NONE',  ( -0.000000000000000000, 1.000000000000000000, -0.000000000000000000 ) ) ;
#68555=CARTESIAN_POINT ( 'NONE',  ( 11.84999999999990727, 2.500000000000000000, -2.511473670974877948 ) ) ;
#68556=FACE_BOUND ( 'NONE', #128911, .T. ) ;
#68557=DIRECTION ( 'NONE',  ( 0.000000000000000000, 1.000000000000000000, 0.000000000000000000 ) ) ;
#68559=CONICAL_SURFACE ( 'NONE', #112397, 0.09999999999999982514, 0.003490658503988666988 ) ;
#68561=CARTESIAN_POINT ( 'NONE',  ( -6.250000000000015987, 12.50000000000000000, 5.737276932171707422 ) ) ;
#68562=ADVANCED_FACE ( 'NONE', ( #112149 ), #13813, .T. ) ;
#68563=AXIS2_PLACEMENT_3D ( 'NONE', #82536, #113264, #1367 ) ;
#68565=DIRECTION ( 'NONE',  ( -4.274815082592931898E-19, -0.9999939076577903929, -0.003490651415223739937 ) ) ;
#68566=DIRECTION ( 'NONE',  ( -0.000000000000000000, -1.000000000000000000, -0.000000000000000000 ) ) ;
#68567=VECTOR ( 'NONE', #36083, 1000.000000000000000 ) ;
#68568=CARTESIAN_POINT ( 'NONE',  ( -10.60000000000000142, 2.500000000000000000, 3.983716857408420964 ) ) ;
#68569=ORIENTED_EDGE ( 'NONE', *, *, #88887, .T. ) ;
#68570=EDGE_LOOP ( 'NONE', ( #68290, #22520, #116765, #15647 ) ) ;
#68571=ORIENTED_EDGE ( 'NONE', *, *, #39379, .F. ) ;
#68572=EDGE_LOOP ( 'NONE', ( #102576, #127057, #4769, #61846 ) ) ;
#68573=EDGE_CURVE ( 'NONE', #63096, #113352, #32325, .T. ) ;
#68574=AXIS2_PLACEMENT_3D ( 'NONE', #19908, #128591, #88636 ) ;
#68575=DIRECTION ( 'NONE',  ( 0.000000000000000000, 0.000000000000000000, -1.000000000000000000 ) ) ;
#68576=DIRECTION ( 'NONE',  ( 0.000000000000000000, 0.000000000000000000, 1.000000000000000000 ) ) ;
#68577=ADVANCED_FACE ( 'NONE', ( #22500 ), #24408, .T. ) ;
#68578=FACE_BOUND ( 'NONE', #116888, .T. ) ;
#68579=FACE_OUTER_BOUND ( 'NONE', #4428, .T. ) ;
#68580=VECTOR ( 'NONE', #108486, 1000.000000000000000 ) ;
#68581=CIRCLE ( 'NONE', #37212, 0.1000000000000002554 ) ;
#68583=DIRECTION ( 'NONE',  ( -0.000000000000000000, -1.000000000000000000, -0.000000000000000000 ) ) ;
#68584=DIRECTION ( 'NONE',  ( -0.000000000000000000, -1.000000000000000000, -0.000000000000000000 ) ) ;
#68585=EDGE_CURVE ( 'NONE', #21407, #75499, #92494, .T. ) ;
#68586=CARTESIAN_POINT ( 'NONE',  ( -5.400000000000019895, 12.50000000000000000, -0.6928203230275541413 ) ) ;
#68587=FACE_OUTER_BOUND ( 'NONE', #46973, .T. ) ;
#68588=VECTOR ( 'NONE', #93753, 1000.000000000000000 ) ;
#68589=VERTEX_POINT ( 'NONE', #84621 ) ;
#68590=AXIS2_PLACEMENT_3D ( 'NONE', #42581, #2615, #113216 ) ;
#68591=LINE ( 'NONE', #7075, #93128 ) ;
#68592=ORIENTED_EDGE ( 'NONE', *, *, #103539, .T. ) ;
#68594=FACE_OUTER_BOUND ( 'NONE', #24738, .T. ) ;
#68595=CARTESIAN_POINT ( 'NONE',  ( -3.150000000000029665, 12.50000000000000000, 6.841600689897072485 ) ) ;
#68596=AXIS2_PLACEMENT_3D ( 'NONE', #83895, #82633, #54437 ) ;
#68597=ORIENTED_EDGE ( 'NONE', *, *, #66576, .F. ) ;
#68598=LINE ( 'NONE', #118994, #5024 ) ;
#68599=DIRECTION ( 'NONE',  ( 0.000000000000000000, 0.000000000000000000, -1.000000000000000000 ) ) ;
#68600=VERTEX_POINT ( 'NONE', #113431 ) ;
#68601=CARTESIAN_POINT ( 'NONE',  ( 8.149999999999923972, 12.50000000000000000, -6.148780366869526226 ) ) ;
#68602=ORIENTED_EDGE ( 'NONE', *, *, #94674, .T. ) ;
#68603=AXIS2_PLACEMENT_3D ( 'NONE', #110438, #52175, #40441 ) ;
#68604=CARTESIAN_POINT ( 'NONE',  ( -6.249999999999984901, 12.50000000000000000, -6.495190528383302464 ) ) ;
#68605=ORIENTED_EDGE ( 'NONE', *, *, #2129, .F. ) ;
#68607=FACE_BOUND ( 'NONE', #89198, .T. ) ;
#68608=ADVANCED_FACE ( 'NONE', ( #64331 ), #55163, .T. ) ;
#68609=VECTOR ( 'NONE', #11664, 1000.000000000000000 ) ;
#68610=ORIENTED_EDGE ( 'NONE', *, *, #36480, .T. ) ;
#68612=ORIENTED_EDGE ( 'NONE', *, *, #101872, .F. ) ;
#68614=DIRECTION ( 'NONE',  ( 0.000000000000000000, 1.000000000000000000, 0.000000000000000000 ) ) ;
#68615=DIRECTION ( 'NONE',  ( 0.000000000000000000, 1.000000000000000000, 0.000000000000000000 ) ) ;
#68616=DIRECTION ( 'NONE',  ( 0.000000000000000000, 0.000000000000000000, 1.000000000000000000 ) ) ;
#68618=EDGE_CURVE ( 'NONE', #13662, #3435, #72421, .T. ) ;
#68619=DIRECTION ( 'NONE',  ( 0.000000000000000000, -0.9999939076577903929, 0.003490651415223739937 ) ) ;
#68620=EDGE_CURVE ( 'NONE', #88669, #118375, #59771, .T. ) ;
#68621=ORIENTED_EDGE ( 'NONE', *, *, #74565, .F. ) ;
#68623=EDGE_LOOP ( 'NONE', ( #57633, #87079, #62610, #46122 ) ) ;
#68624=DIRECTION ( 'NONE',  ( 0.000000000000000000, 0.000000000000000000, -1.000000000000000000 ) ) ;
#68625=DIRECTION ( 'NONE',  ( 0.000000000000000000, 0.000000000000000000, 1.000000000000000000 ) ) ;
#68626=ADVANCED_FACE ( 'NONE', ( #14571 ), #128881, .T. ) ;
#68627=DIRECTION ( 'NONE',  ( -0.000000000000000000, -1.000000000000000000, -0.000000000000000000 ) ) ;
#68628=AXIS2_PLACEMENT_3D ( 'NONE', #32222, #119938, #72132 ) ;
#68629=EDGE_LOOP ( 'NONE', ( #118009, #41440, #68932, #93557 ) ) ;
#68630=ORIENTED_EDGE ( 'NONE', *, *, #107475, .F. ) ;
#68631=EDGE_CURVE ( 'NONE', #101262, #96780, #54501, .T. ) ;
#68632=EDGE_LOOP ( 'NONE', ( #125516, #36767, #94941, #22364 ) ) ;
#68633=ADVANCED_FACE ( 'NONE', ( #45350 ), #122597, .T. ) ;
#68634=DIRECTION ( 'NONE',  ( 0.000000000000000000, 0.000000000000000000, -1.000000000000000000 ) ) ;
#68635=DIRECTION ( 'NONE',  ( -0.000000000000000000, 1.000000000000000000, -0.000000000000000000 ) ) ;
#68638=CARTESIAN_POINT ( 'NONE',  ( -12.04999999999999538, 12.50000000000000000, 2.230156782645134950 ) ) ;
#68639=CARTESIAN_POINT ( 'NONE',  ( 1.049999999999954081, 2.500000000000000000, -6.048780366869526581 ) ) ;
#68640=CIRCLE ( 'NONE', #118815, 0.06509327318403743123 ) ;
#68641=DIRECTION ( 'NONE',  ( 0.000000000000000000, 0.000000000000000000, 1.000000000000000000 ) ) ;
#68642=DIRECTION ( 'NONE',  ( 0.000000000000000000, 0.000000000000000000, 1.000000000000000000 ) ) ;
#68643=DIRECTION ( 'NONE',  ( 0.000000000000000000, 0.000000000000000000, 1.000000000000000000 ) ) ;
#68644=EDGE_CURVE ( 'NONE', #103825, #65666, #103730, .T. ) ;
#68645=DIRECTION ( 'NONE',  ( 0.000000000000000000, 0.000000000000000000, -1.000000000000000000 ) ) ;
#68646=EDGE_CURVE ( 'NONE', #49853, #42996, #124655, .T. ) ;
#68647=VECTOR ( 'NONE', #55109, 1000.000000000000000 ) ;
#68648=ORIENTED_EDGE ( 'NONE', *, *, #111733, .F. ) ;
#68649=AXIS2_PLACEMENT_3D ( 'NONE', #5200, #63502, #4538 ) ;
#68650=EDGE_LOOP ( 'NONE', ( #40347, #129468 ) ) ;
#68651=CIRCLE ( 'NONE', #83237, 0.06509327318403745899 ) ;
#68652=CARTESIAN_POINT ( 'NONE',  ( 4.349999999999941025, 12.50000000000000000, -6.148780366869526226 ) ) ;
#68653=CARTESIAN_POINT ( 'NONE',  ( 10.39999999999991154, 12.50000000000000000, -5.022947341949754119 ) ) ;
#68654=ORIENTED_EDGE ( 'NONE', *, *, #69040, .T. ) ;
#68655=VERTEX_POINT ( 'NONE', #4740 ) ;
#68657=DIRECTION ( 'NONE',  ( 0.000000000000000000, 0.000000000000000000, 1.000000000000000000 ) ) ;
#68658=CARTESIAN_POINT ( 'NONE',  ( -11.64999999999999680, 12.50000000000000000, 5.802370205355744659 ) ) ;
#68659=VECTOR ( 'NONE', #57461, 1000.000000000000000 ) ;
#68660=CARTESIAN_POINT ( 'NONE',  ( 8.349999999999923261, 12.50000000000000000, -5.802370205355749988 ) ) ;
#68661=AXIS2_PLACEMENT_3D ( 'NONE', #56274, #5871, #105384 ) ;
#68662=DIRECTION ( 'NONE',  ( -0.000000000000000000, -1.000000000000000000, -0.000000000000000000 ) ) ;
#68663=CARTESIAN_POINT ( 'NONE',  ( 0.3999999999999628852, 2.500000000000000000, -0.5928203230275519431 ) ) ;
#68664=CARTESIAN_POINT ( 'NONE',  ( 6.699999999999928235, 12.50000000000000000, -2.276824562219559311E-15 ) ) ;
#68665=DIRECTION ( 'NONE',  ( 0.000000000000000000, 1.000000000000000000, 0.000000000000000000 ) ) ;
#68666=CIRCLE ( 'NONE', #127178, 0.09999999999999982514 ) ;
#68667=ORIENTED_EDGE ( 'NONE', *, *, #101903, .F. ) ;
#68668=EDGE_LOOP ( 'NONE', ( #48118, #55462, #10343, #62159 ) ) ;
#68670=CONICAL_SURFACE ( 'NONE', #120898, 0.09999999999999982514, 0.003490658503988666988 ) ;
#68671=ORIENTED_EDGE ( 'NONE', *, *, #72415, .F. ) ;
#68672=ORIENTED_EDGE ( 'NONE', *, *, #103174, .T. ) ;
#68673=CARTESIAN_POINT ( 'NONE',  ( 12.89999999999990266, 12.50000000000000000, -5.022947341949754119 ) ) ;
#68674=CARTESIAN_POINT ( 'NONE',  ( -5.200000000000020606, 12.50000000000000000, 3.983716857408420964 ) ) ;
#68675=CIRCLE ( 'NONE', #22639, 0.06509327318403745899 ) ;
#68676=VERTEX_POINT ( 'NONE', #123256 ) ;
#68677=DIRECTION ( 'NONE',  ( 0.000000000000000000, -0.9999939076577903929, 0.003490651415223739937 ) ) ;
#68678=EDGE_CURVE ( 'NONE', #62565, #59648, #76533, .T. ) ;
#68679=CARTESIAN_POINT ( 'NONE',  ( -3.350000000000031619, 2.500000000000000000, -7.188010851410854052 ) ) ;
#68680=EDGE_CURVE ( 'NONE', #81291, #49092, #30576, .T. ) ;
#68681=DIRECTION ( 'NONE',  ( -4.274815082592931898E-19, -0.9999939076577903929, -0.003490651415223739937 ) ) ;
#68682=DIRECTION ( 'NONE',  ( 0.000000000000000000, 0.000000000000000000, 1.000000000000000000 ) ) ;
#68683=VERTEX_POINT ( 'NONE', #85885 ) ;
#68684=DIRECTION ( 'NONE',  ( 0.000000000000000000, 0.000000000000000000, 1.000000000000000000 ) ) ;
#68685=CIRCLE ( 'NONE', #54029, 0.06509327318403745899 ) ;
#68686=DIRECTION ( 'NONE',  ( 0.000000000000000000, 0.000000000000000000, 1.000000000000000000 ) ) ;
#68687=ORIENTED_EDGE ( 'NONE', *, *, #52846, .F. ) ;
#68688=AXIS2_PLACEMENT_3D ( 'NONE', #58419, #48589, #88496 ) ;
#68689=EDGE_LOOP ( 'NONE', ( #12851, #18348, #29684, #40073 ) ) ;
#68690=ORIENTED_EDGE ( 'NONE', *, *, #2421, .F. ) ;
#68691=ORIENTED_EDGE ( 'NONE', *, *, #104752, .T. ) ;
#68692=CARTESIAN_POINT ( 'NONE',  ( -5.400000000000019895, 2.500000000000000000, 3.537306695894645081 ) ) ;
#68693=CIRCLE ( 'NONE', #122991, 0.1000000000000002554 ) ;
#68694=CARTESIAN_POINT ( 'NONE',  ( -12.49999999999995914, 2.500000000000000000, -4.330127018922198978 ) ) ;
#68695=CIRCLE ( 'NONE', #45727, 0.06509327318403745899 ) ;
#68696=EDGE_LOOP ( 'NONE', ( #56910, #22823, #108614, #123225 ) ) ;
#68697=DIRECTION ( 'NONE',  ( -4.274815082592931898E-19, -0.9999939076577903929, -0.003490651415223739937 ) ) ;
#68698=CARTESIAN_POINT ( 'NONE',  ( 1.249999999999950262, 12.50000000000000000, 7.188010851410848723 ) ) ;
#68699=AXIS2_PLACEMENT_3D ( 'NONE', #93389, #23337, #65187 ) ;
#68701=CARTESIAN_POINT ( 'NONE',  ( -4.550000000000022915, 2.500000000000000000, 6.395190528383296602 ) ) ;
#68702=ORIENTED_EDGE ( 'NONE', *, *, #63218, .F. ) ;
#68704=AXIS2_PLACEMENT_3D ( 'NONE', #17493, #65964, #16200 ) ;
#68705=CARTESIAN_POINT ( 'NONE',  ( -10.40000000000000213, 2.500000000000000000, -0.1000000000000022815 ) ) ;
#68707=ORIENTED_EDGE ( 'NONE', *, *, #55152, .T. ) ;
#68708=DIRECTION ( 'NONE',  ( -0.000000000000000000, 1.000000000000000000, -0.000000000000000000 ) ) ;
#68709=DIRECTION ( 'NONE',  ( 0.000000000000000000, 0.000000000000000000, 1.000000000000000000 ) ) ;
#68710=FACE_BOUND ( 'NONE', #20429, .T. ) ;
#68711=DIRECTION ( 'NONE',  ( -0.000000000000000000, 1.000000000000000000, -0.000000000000000000 ) ) ;
#68712=DIRECTION ( 'NONE',  ( -0.000000000000000000, 1.000000000000000000, -0.000000000000000000 ) ) ;
#68713=CARTESIAN_POINT ( 'NONE',  ( -0.8000000000000376810, 2.500000000000000000, -4.230127018922201998 ) ) ;
#68714=EDGE_CURVE ( 'NONE', #114690, #22290, #57747, .T. ) ;
#68715=AXIS2_PLACEMENT_3D ( 'NONE', #25425, #37215, #97405 ) ;
#68716=ORIENTED_EDGE ( 'NONE', *, *, #6553, .F. ) ;
#68717=LINE ( 'NONE', #100126, #19134 ) ;
#68718=CARTESIAN_POINT ( 'NONE',  ( -12.09999999999999609, 2.500000000000000000, 4.330127018922196314 ) ) ;
#68719=DIRECTION ( 'NONE',  ( 0.000000000000000000, 0.000000000000000000, 1.000000000000000000 ) ) ;
#68720=DIRECTION ( 'NONE',  ( 0.000000000000000000, 1.000000000000000000, 0.000000000000000000 ) ) ;
#68721=EDGE_LOOP ( 'NONE', ( #8104, #61240 ) ) ;
#68722=ADVANCED_FACE ( 'NONE', ( #37464 ), #99522, .T. ) ;
#68723=PLANE ( 'NONE',  #11456 ) ;
#68724=AXIS2_PLACEMENT_3D ( 'NONE', #75279, #115178, #25523 ) ;
#68725=AXIS2_PLACEMENT_3D ( 'NONE', #93622, #36655, #54975 ) ;
#68726=CARTESIAN_POINT ( 'NONE',  ( -6.700000000000019718, 2.500000000000000000, -4.230127018922201998 ) ) ;
#68727=AXIS2_PLACEMENT_3D ( 'NONE', #82341, #120956, #122262 ) ;
#68728=EDGE_LOOP ( 'NONE', ( #72480, #17896, #61350, #49152 ) ) ;
#68729=ORIENTED_EDGE ( 'NONE', *, *, #121219, .T. ) ;
#68731=FACE_OUTER_BOUND ( 'NONE', #58587, .T. ) ;
#68732=DIRECTION ( 'NONE',  ( -0.000000000000000000, -1.000000000000000000, -0.000000000000000000 ) ) ;
#68733=EDGE_CURVE ( 'NONE', #36724, #96060, #59837, .T. ) ;
#68734=FACE_BOUND ( 'NONE', #112741, .T. ) ;
#68735=CARTESIAN_POINT ( 'NONE',  ( 11.74779829714320378, -2.500000000000001776, -7.682567038344338073 ) ) ;
#68736=VECTOR ( 'NONE', #64337, 1000.000000000000000 ) ;
#68737=CIRCLE ( 'NONE', #83425, 0.06509327318403745899 ) ;
#68738=VECTOR ( 'NONE', #79599, 1000.000000000000000 ) ;
#68739=ORIENTED_EDGE ( 'NONE', *, *, #124329, .F. ) ;
#68740=DIRECTION ( 'NONE',  ( 0.000000000000000000, 0.000000000000000000, 1.000000000000000000 ) ) ;
#68741=VERTEX_POINT ( 'NONE', #106198 ) ;
#68742=EDGE_LOOP ( 'NONE', ( #23918, #67638 ) ) ;
#68743=DIRECTION ( 'NONE',  ( 0.000000000000000000, 0.000000000000000000, 1.000000000000000000 ) ) ;
#68744=EDGE_CURVE ( 'NONE', #86614, #32914, #1300, .T. ) ;
#68747=DIRECTION ( 'NONE',  ( -0.000000000000000000, 1.000000000000000000, -0.000000000000000000 ) ) ;
#68748=CARTESIAN_POINT ( 'NONE',  ( -2.100000000000033840, 2.500000000000000000, 4.922947341949748257 ) ) ;
#68749=AXIS2_PLACEMENT_3D ( 'NONE', #59536, #60168, #79787 ) ;
#68750=PLANE ( 'NONE',  #10993 ) ;
#68751=DIRECTION ( 'NONE',  ( 0.000000000000000000, -0.9999939076577903929, 0.003490651415223739937 ) ) ;
#68752=EDGE_LOOP ( 'NONE', ( #32428, #26911 ) ) ;
#68753=DIRECTION ( 'NONE',  ( -0.000000000000000000, -1.000000000000000000, -0.000000000000000000 ) ) ;
#68754=CARTESIAN_POINT ( 'NONE',  ( 8.349999999999919709, 2.500000000000000000, -2.065063509461102065 ) ) ;
#68755=CARTESIAN_POINT ( 'NONE',  ( -2.050000000000033129, 12.50000000000000000, 6.495190528383297135 ) ) ;
#68756=AXIS2_PLACEMENT_3D ( 'NONE', #90393, #100864, #30226 ) ;
#68757=FACE_OUTER_BOUND ( 'NONE', #74935, .T. ) ;
#68758=ORIENTED_EDGE ( 'NONE', *, *, #37457, .F. ) ;
#68759=ORIENTED_EDGE ( 'NONE', *, *, #15834, .F. ) ;
#68760=LINE ( 'NONE', #108688, #116157 ) ;
#68761=ORIENTED_EDGE ( 'NONE', *, *, #70740, .F. ) ;
#68762=DIRECTION ( 'NONE',  ( 0.000000000000000000, -0.9999939076577903929, 0.003490651415223739937 ) ) ;
#68763=CARTESIAN_POINT ( 'NONE',  ( 87.50000000000001421, -6.099025433955698183, -4.412011999988000532 ) ) ;
#68764=EDGE_CURVE ( 'NONE', #95676, #6638, #95734, .T. ) ;
#68765=CARTESIAN_POINT ( 'NONE',  ( -10.40000000000000213, 2.500000000000000000, -0.5928203230275541635 ) ) ;
#68766=DIRECTION ( 'NONE',  ( -0.000000000000000000, 1.000000000000000000, -0.000000000000000000 ) ) ;
#68767=ORIENTED_EDGE ( 'NONE', *, *, #60584, .T. ) ;
#68768=AXIS2_PLACEMENT_3D ( 'NONE', #84772, #106342, #93951 ) ;
#68769=DIRECTION ( 'NONE',  ( -0.000000000000000000, 1.000000000000000000, -0.000000000000000000 ) ) ;
#68770=LINE ( 'NONE', #58963, #14629 ) ;
#68771=CARTESIAN_POINT ( 'NONE',  ( 10.59999999999990905, 2.500000000000000000, 3.983716857408420076 ) ) ;
#68773=CARTESIAN_POINT ( 'NONE',  ( -11.64999999999999680, 12.50000000000000000, 2.165063509461097713 ) ) ;
#68774=EDGE_CURVE ( 'NONE', #93079, #74476, #41043, .T. ) ;
#68775=VECTOR ( 'NONE', #63824, 1000.000000000000000 ) ;
#68776=DIRECTION ( 'NONE',  ( -4.274815082592931898E-19, -0.9999939076577903929, -0.003490651415223739937 ) ) ;
#68777=EDGE_CURVE ( 'NONE', #78711, #127931, #68198, .T. ) ;
#68778=CIRCLE ( 'NONE', #52073, 0.09999999999999982514 ) ;
#68779=ORIENTED_EDGE ( 'NONE', *, *, #117054, .F. ) ;
#68780=EDGE_LOOP ( 'NONE', ( #38734, #107160, #61740, #7937 ) ) ;
#68781=DIRECTION ( 'NONE',  ( 0.000000000000000000, 0.000000000000000000, -1.000000000000000000 ) ) ;
#68782=ORIENTED_EDGE ( 'NONE', *, *, #118786, .T. ) ;
#68783=DIRECTION ( 'NONE',  ( 0.000000000000000000, 0.000000000000000000, 1.000000000000000000 ) ) ;
#68784=EDGE_CURVE ( 'NONE', #44544, #2580, #7977, .T. ) ;
#68785=EDGE_LOOP ( 'NONE', ( #18210, #118059 ) ) ;
#68786=ORIENTED_EDGE ( 'NONE', *, *, #92089, .F. ) ;
#68787=EDGE_CURVE ( 'NONE', #94775, #36193, #61955, .T. ) ;
#68788=ORIENTED_EDGE ( 'NONE', *, *, #100547, .T. ) ;
#68789=CIRCLE ( 'NONE', #79273, 0.06509327318403745899 ) ;
#68790=ADVANCED_FACE ( 'NONE', ( #6039 ), #26351, .T. ) ;
#68791=DIRECTION ( 'NONE',  ( 0.000000000000000000, 0.000000000000000000, 1.000000000000000000 ) ) ;
#68792=ADVANCED_FACE ( 'NONE', ( #115336 ), #53551, .T. ) ;
#68793=LINE ( 'NONE', #108713, #12980 ) ;
#68794=DIRECTION ( 'NONE',  ( 0.000000000000000000, 0.000000000000000000, 1.000000000000000000 ) ) ;
#68795=CIRCLE ( 'NONE', #85517, 0.06509327318403745899 ) ;
#68796=CONICAL_SURFACE ( 'NONE', #26945, 0.09999999999999982514, 0.003490658503988666988 ) ;
#68797=EDGE_CURVE ( 'NONE', #48784, #80079, #5498, .T. ) ;
#68798=CARTESIAN_POINT ( 'NONE',  ( -5.200000000000025935, 2.500000000000000000, -3.983716857408426293 ) ) ;
#68800=LINE ( 'NONE', #108718, #70625 ) ;
#68801=CARTESIAN_POINT ( 'NONE',  ( -12.09999999999999609, 2.500000000000000000, -3.637306695894647390 ) ) ;
#68802=AXIS2_PLACEMENT_3D ( 'NONE', #1616, #50108, #30467 ) ;
#68803=DIRECTION ( 'NONE',  ( 0.000000000000000000, 0.000000000000000000, 1.000000000000000000 ) ) ;
#68804=ADVANCED_FACE ( 'NONE', ( #76089 ), #15960, .T. ) ;
#68805=ORIENTED_EDGE ( 'NONE', *, *, #47965, .T. ) ;
#68806=CIRCLE ( 'NONE', #123195, 0.06509327318403745899 ) ;
#68807=CIRCLE ( 'NONE', #77217, 0.06509327318403745899 ) ;
#68808=EDGE_LOOP ( 'NONE', ( #65558, #16371 ) ) ;
#68809=ORIENTED_EDGE ( 'NONE', *, *, #74650, .F. ) ;
#68810=CARTESIAN_POINT ( 'NONE',  ( 4.549999999999937650, 2.500000000000000000, 2.165063509461097713 ) ) ;
#68811=ORIENTED_EDGE ( 'NONE', *, *, #76671, .F. ) ;
#68812=ORIENTED_EDGE ( 'NONE', *, *, #34477, .T. ) ;
#68813=CARTESIAN_POINT ( 'NONE',  ( -4.800000000000028244, 2.500000000000000000, -4.083716857408426826 ) ) ;
#68814=CARTESIAN_POINT ( 'NONE',  ( 2.499999999999983569, 2.500000000000000000, -4.430127018922202176 ) ) ;
#68815=DIRECTION ( 'NONE',  ( 0.000000000000000000, 1.000000000000000000, 0.000000000000000000 ) ) ;
#68816=FACE_OUTER_BOUND ( 'NONE', #118751, .T. ) ;
#68817=CARTESIAN_POINT ( 'NONE',  ( -10.80000000000000071, 2.500000000000000000, 4.330127018922196314 ) ) ;
#68818=AXIS2_PLACEMENT_3D ( 'NONE', #128524, #97734, #66968 ) ;
#68819=ORIENTED_EDGE ( 'NONE', *, *, #127672, .T. ) ;
#68820=EDGE_LOOP ( 'NONE', ( #87518, #27928, #47441, #6720 ) ) ;
#68821=CIRCLE ( 'NONE', #60533, 0.06509327318403745899 ) ;
#68822=FACE_OUTER_BOUND ( 'NONE', #43767, .T. ) ;
#68823=AXIS2_PLACEMENT_3D ( 'NONE', #92834, #20220, #91535 ) ;
#68824=ORIENTED_EDGE ( 'NONE', *, *, #116660, .T. ) ;
#68825=DIRECTION ( 'NONE',  ( 0.000000000000000000, -0.9999939076577903929, 0.003490651415223739937 ) ) ;
#68826=ORIENTED_EDGE ( 'NONE', *, *, #95085, .T. ) ;
#68827=ORIENTED_EDGE ( 'NONE', *, *, #38307, .T. ) ;
#68828=CARTESIAN_POINT ( 'NONE',  ( -6.249999999999981348, 2.500000000000000000, 6.395190528383296602 ) ) ;
#68829=CIRCLE ( 'NONE', #27073, 0.06509327318403745899 ) ;
#68830=CARTESIAN_POINT ( 'NONE',  ( -1.450000000000036371, 2.500000000000000000, 6.941600689897073018 ) ) ;
#68831=CIRCLE ( 'NONE', #123226, 0.06509327318403743123 ) ;
#68832=CARTESIAN_POINT ( 'NONE',  ( 2.699999999999946443, 2.500000000000000000, -3.883716857408426648 ) ) ;
#68833=ADVANCED_FACE ( 'NONE', ( #35530 ), #7553, .T. ) ;
#68834=DIRECTION ( 'NONE',  ( -0.000000000000000000, 1.000000000000000000, -0.000000000000000000 ) ) ;
#68835=CARTESIAN_POINT ( 'NONE',  ( 4.999999999999969802, 2.500000000000000000, 4.330127018922196314 ) ) ;
#68836=ORIENTED_EDGE ( 'NONE', *, *, #120806, .F. ) ;
#68837=CARTESIAN_POINT ( 'NONE',  ( -6.250000000000017764, 2.500000000000000000, 7.088010851410848190 ) ) ;
#68838=FACE_OUTER_BOUND ( 'NONE', #29422, .T. ) ;
#68839=CARTESIAN_POINT ( 'NONE',  ( -13.54999999999999005, 12.50000000000000000, 2.511473670974877503 ) ) ;
#68840=DIRECTION ( 'NONE',  ( 0.000000000000000000, 1.000000000000000000, 0.000000000000000000 ) ) ;
#68841=VECTOR ( 'NONE', #59902, 1000.000000000000000 ) ;
#68842=DIRECTION ( 'NONE',  ( 0.000000000000000000, 0.000000000000000000, 1.000000000000000000 ) ) ;
#68843=ADVANCED_FACE ( 'NONE', ( #46617 ), #26363, .T. ) ;
#68844=AXIS2_PLACEMENT_3D ( 'NONE', #82715, #64343, #72250 ) ;
#68845=EDGE_LOOP ( 'NONE', ( #66793, #73763 ) ) ;
#68846=AXIS2_PLACEMENT_3D ( 'NONE', #27027, #17162, #87855 ) ;
#68847=ORIENTED_EDGE ( 'NONE', *, *, #62911, .F. ) ;
#68848=CARTESIAN_POINT ( 'NONE',  ( 14.14999999999989733, 2.500000000000000000, 1.472243186433545459 ) ) ;
#68849=ORIENTED_EDGE ( 'NONE', *, *, #5210, .T. ) ;
#68850=DIRECTION ( 'NONE',  ( 0.000000000000000000, 1.000000000000000000, 0.000000000000000000 ) ) ;
#68851=LINE ( 'NONE', #98959, #41858 ) ;
#68852=AXIS2_PLACEMENT_3D ( 'NONE', #98600, #38440, #8298 ) ;
#68853=ORIENTED_EDGE ( 'NONE', *, *, #41582, .T. ) ;
#68855=DIRECTION ( 'NONE',  ( -0.000000000000000000, 1.000000000000000000, -0.000000000000000000 ) ) ;
#68856=CARTESIAN_POINT ( 'NONE',  ( -8.950000000000009948, 2.500000000000000000, -6.841600689897072485 ) ) ;
#68857=CARTESIAN_POINT ( 'NONE',  ( -8.550000000000013145, 2.500000000000000000, -6.741600689897072840 ) ) ;
#68858=ORIENTED_EDGE ( 'NONE', *, *, #101448, .F. ) ;
#68859=CARTESIAN_POINT ( 'NONE',  ( -3.750000000000027978, 2.500000000000000000, 7.188010851410848723 ) ) ;
#68860=ORIENTED_EDGE ( 'NONE', *, *, #111943, .T. ) ;
#68861=DIRECTION ( 'NONE',  ( -0.000000000000000000, -1.000000000000000000, -0.000000000000000000 ) ) ;
#68862=CIRCLE ( 'NONE', #22912, 0.06509327318403745899 ) ;
#68863=FACE_OUTER_BOUND ( 'NONE', #103316, .T. ) ;
#68864=CARTESIAN_POINT ( 'NONE',  ( 3.949999999999938005, 12.50000000000000000, 6.841600689897072485 ) ) ;
#68865=EDGE_CURVE ( 'NONE', #30644, #103084, #36818, .T. ) ;
#68866=ORIENTED_EDGE ( 'NONE', *, *, #49073, .T. ) ;
#68867=CARTESIAN_POINT ( 'NONE',  ( 13.94999999999989804, 2.500000000000000000, 1.818653347947321475 ) ) ;
#68868=ORIENTED_EDGE ( 'NONE', *, *, #113293, .F. ) ;
#68870=AXIS2_PLACEMENT_3D ( 'NONE', #19862, #99714, #1491 ) ;
#68871=DIRECTION ( 'NONE',  ( 0.000000000000000000, -0.9999939076577903929, 0.003490651415223739937 ) ) ;
#68872=DIRECTION ( 'NONE',  ( 0.000000000000000000, 1.000000000000000000, 0.000000000000000000 ) ) ;
#68873=ORIENTED_EDGE ( 'NONE', *, *, #98744, .T. ) ;
#68874=EDGE_CURVE ( 'NONE', #120570, #124699, #70276, .T. ) ;
#68875=LINE ( 'NONE', #8019, #11264 ) ;
#68876=CARTESIAN_POINT ( 'NONE',  ( 12.49999999999990585, 12.50000000000000000, -4.957854068765716882 ) ) ;
#68877=AXIS2_PLACEMENT_3D ( 'NONE', #166, #30315, #826 ) ;
#68878=EDGE_CURVE ( 'NONE', #66105, #35393, #24296, .T. ) ;
#68879=ORIENTED_EDGE ( 'NONE', *, *, #125522, .T. ) ;
#68880=EDGE_CURVE ( 'NONE', #31883, #100718, #108753, .T. ) ;
#68881=DIRECTION ( 'NONE',  ( 0.000000000000000000, 0.000000000000000000, 1.000000000000000000 ) ) ;
#68882=EDGE_CURVE ( 'NONE', #13198, #39312, #30671, .T. ) ;
#68883=ORIENTED_EDGE ( 'NONE', *, *, #10967, .F. ) ;
#68884=CARTESIAN_POINT ( 'NONE',  ( 2.499999999999947153, 2.500000000000000000, 3.637306695894644726 ) ) ;
#68885=VECTOR ( 'NONE', #61774, 1000.000000000000000 ) ;
#68886=CIRCLE ( 'NONE', #70955, 0.09999999999999982514 ) ;
#68887=EDGE_LOOP ( 'NONE', ( #62423, #27135, #101424, #52166 ) ) ;
#68889=DIRECTION ( 'NONE',  ( 0.000000000000000000, 1.000000000000000000, 0.000000000000000000 ) ) ;
#68890=EDGE_CURVE ( 'NONE', #46014, #98786, #5580, .T. ) ;
#68891=ORIENTED_EDGE ( 'NONE', *, *, #49644, .F. ) ;
#68892=ORIENTED_EDGE ( 'NONE', *, *, #16446, .F. ) ;
#68893=ADVANCED_FACE ( 'NONE', ( #68838 ), #66143, .T. ) ;
#68894=DIRECTION ( 'NONE',  ( -4.274815082592931898E-19, -0.9999939076577903929, -0.003490651415223739937 ) ) ;
#68895=FACE_OUTER_BOUND ( 'NONE', #126146, .T. ) ;
#68896=VERTEX_POINT ( 'NONE', #21024 ) ;
#68897=DIRECTION ( 'NONE',  ( 0.000000000000000000, -0.000000000000000000, 1.000000000000000000 ) ) ;
#68898=CARTESIAN_POINT ( 'NONE',  ( 2.299999999999948752, 12.50000000000000000, 0.3464101615137735735 ) ) ;
#68899=FACE_OUTER_BOUND ( 'NONE', #62459, .T. ) ;
#68901=CONICAL_SURFACE ( 'NONE', #38406, 0.1000000000000000472, 0.003490658503988666988 ) ;
#68902=CARTESIAN_POINT ( 'NONE',  ( 8.949999999999919353, 12.50000000000000000, 2.511473670974873507 ) ) ;
#68903=DIRECTION ( 'NONE',  ( 0.000000000000000000, 0.000000000000000000, -1.000000000000000000 ) ) ;
#68904=DIRECTION ( 'NONE',  ( 0.000000000000000000, 0.000000000000000000, 1.000000000000000000 ) ) ;
#68905=AXIS2_PLACEMENT_3D ( 'NONE', #82054, #113453, #112172 ) ;
#68906=CIRCLE ( 'NONE', #54250, 0.09999999999999982514 ) ;
#68907=EDGE_LOOP ( 'NONE', ( #37960, #84185, #124708, #17683 ) ) ;
#68908=EDGE_LOOP ( 'NONE', ( #122644, #54350, #72660, #13486 ) ) ;
#68909=VERTEX_POINT ( 'NONE', #60947 ) ;
#68910=ORIENTED_EDGE ( 'NONE', *, *, #50875, .T. ) ;
#68911=DIRECTION ( 'NONE',  ( 0.000000000000000000, 0.000000000000000000, 1.000000000000000000 ) ) ;
#68912=DIRECTION ( 'NONE',  ( 0.000000000000000000, 1.000000000000000000, 0.000000000000000000 ) ) ;
#68913=CARTESIAN_POINT ( 'NONE',  ( 12.89999999999989910, 12.50000000000000000, -0.6277270498435167934 ) ) ;
#68914=ORIENTED_EDGE ( 'NONE', *, *, #17539, .T. ) ;
#68915=FACE_BOUND ( 'NONE', #28195, .T. ) ;
#68916=EDGE_LOOP ( 'NONE', ( #95239, #55429, #13224, #100612 ) ) ;
#68917=CARTESIAN_POINT ( 'NONE',  ( -12.29999999999999716, 2.500000000000000000, -4.083716857408424161 ) ) ;
#68918=CARTESIAN_POINT ( 'NONE',  ( 8.949999999999919353, 2.500000000000000000, 2.411473670974873862 ) ) ;
#68919=CIRCLE ( 'NONE', #125073, 0.06509327318403745899 ) ;
#68920=CIRCLE ( 'NONE', #106295, 0.1000000000000002554 ) ;
#68921=CIRCLE ( 'NONE', #117017, 0.06509327318403745899 ) ;
#68922=CARTESIAN_POINT ( 'NONE',  ( -14.14999999999998614, 2.500000000000000000, -2.265063509461099578 ) ) ;
#68923=DIRECTION ( 'NONE',  ( 0.000000000000000000, 0.000000000000000000, -1.000000000000000000 ) ) ;
#68924=DIRECTION ( 'NONE',  ( 0.000000000000000000, 0.000000000000000000, 1.000000000000000000 ) ) ;
#68925=CARTESIAN_POINT ( 'NONE',  ( -2.900000000000029221, 12.50000000000000000, -5.022947341949754119 ) ) ;
#68926=DIRECTION ( 'NONE',  ( 0.000000000000000000, 0.000000000000000000, 1.000000000000000000 ) ) ;
#68927=DIRECTION ( 'NONE',  ( 0.000000000000000000, 0.000000000000000000, -1.000000000000000000 ) ) ;
#68928=DIRECTION ( 'NONE',  ( -0.000000000000000000, 1.000000000000000000, -0.000000000000000000 ) ) ;
#68929=AXIS2_PLACEMENT_3D ( 'NONE', #103517, #85155, #42688 ) ;
#68930=DIRECTION ( 'NONE',  ( -0.000000000000000000, 1.000000000000000000, -0.000000000000000000 ) ) ;
#68931=EDGE_LOOP ( 'NONE', ( #114893, #17936, #70014, #18044 ) ) ;
#68932=ORIENTED_EDGE ( 'NONE', *, *, #40722, .T. ) ;
#68933=AXIS2_PLACEMENT_3D ( 'NONE', #11881, #41998, #95609 ) ;
#68934=ORIENTED_EDGE ( 'NONE', *, *, #45927, .T. ) ;
#68936=DIRECTION ( 'NONE',  ( 0.000000000000000000, 0.000000000000000000, 1.000000000000000000 ) ) ;
#68937=ADVANCED_FACE ( 'NONE', ( #128434 ), #57853, .T. ) ;
#68938=DIRECTION ( 'NONE',  ( 0.000000000000000000, -0.000000000000000000, 1.000000000000000000 ) ) ;
#68939=EDGE_CURVE ( 'NONE', #26454, #22443, #22349, .T. ) ;
#68940=EDGE_LOOP ( 'NONE', ( #89714, #24745 ) ) ;
#68941=ORIENTED_EDGE ( 'NONE', *, *, #87938, .T. ) ;
#68942=EDGE_LOOP ( 'NONE', ( #124548, #84861 ) ) ;
#68943=ADVANCED_FACE ( 'NONE', ( #51150 ), #78790, .T. ) ;
#68945=CIRCLE ( 'NONE', #20922, 0.1000000000000002554 ) ;
#68946=EDGE_CURVE ( 'NONE', #70149, #32170, #95485, .T. ) ;
#68947=FACE_OUTER_BOUND ( 'NONE', #7244, .T. ) ;
#68949=CARTESIAN_POINT ( 'NONE',  ( -4.400000000000025224, 2.500000000000000000, 3.883716857408420431 ) ) ;
#68950=EDGE_CURVE ( 'NONE', #78428, #80892, #91058, .T. ) ;
#68951=CARTESIAN_POINT ( 'NONE',  ( -9.150000000000009237, 2.500000000000000000, -2.165063509461101710 ) ) ;
#68952=AXIS2_PLACEMENT_3D ( 'NONE', #92449, #32916, #13882 ) ;
#68953=DIRECTION ( 'NONE',  ( 0.000000000000000000, 0.000000000000000000, 1.000000000000000000 ) ) ;
#68954=CARTESIAN_POINT ( 'NONE',  ( -7.300000000000016698, 12.50000000000000000, -4.676537180435978769 ) ) ;
#68955=EDGE_LOOP ( 'NONE', ( #37627, #23666, #24104, #24398 ) ) ;
#68956=CARTESIAN_POINT ( 'NONE',  ( -7.100000000000017408, 2.500000000000000000, -0.6928203230275542523 ) ) ;
#68957=EDGE_CURVE ( 'NONE', #58927, #122539, #49535, .T. ) ;
#68958=ORIENTED_EDGE ( 'NONE', *, *, #122653, .T. ) ;
#68959=ADVANCED_FACE ( 'NONE', ( #71399 ), #9920, .T. ) ;
#68960=ORIENTED_EDGE ( 'NONE', *, *, #97444, .F. ) ;
#68961=ORIENTED_EDGE ( 'NONE', *, *, #101108, .F. ) ;
#68962=CARTESIAN_POINT ( 'NONE',  ( 12.04999999999990834, 2.500000000000000000, 6.595190528383296780 ) ) ;
#68963=VERTEX_POINT ( 'NONE', #88466 ) ;
#68964=ORIENTED_EDGE ( 'NONE', *, *, #110729, .F. ) ;
#68965=EDGE_CURVE ( 'NONE', #5027, #61413, #19072, .T. ) ;
#68966=DIRECTION ( 'NONE',  ( 0.000000000000000000, -0.9999939076577903929, 0.003490651415223739937 ) ) ;
#68967=CARTESIAN_POINT ( 'NONE',  ( 3.949999999999938893, 12.50000000000000000, 6.213873640053558134 ) ) ;
#68968=DIRECTION ( 'NONE',  ( 0.000000000000000000, 1.000000000000000000, 0.000000000000000000 ) ) ;
#68969=DIRECTION ( 'NONE',  ( 0.000000000000000000, 0.000000000000000000, -1.000000000000000000 ) ) ;
#68970=FACE_OUTER_BOUND ( 'NONE', #105400, .T. ) ;
#68971=CIRCLE ( 'NONE', #25059, 0.1000000000000002554 ) ;
#68972=ORIENTED_EDGE ( 'NONE', *, *, #48216, .T. ) ;
#68973=CARTESIAN_POINT ( 'NONE',  ( -5.400000000000023448, 2.500000000000000000, -4.330127018922201643 ) ) ;
#68974=ORIENTED_EDGE ( 'NONE', *, *, #102033, .F. ) ;
#68975=DIRECTION ( 'NONE',  ( 0.000000000000000000, 0.000000000000000000, 1.000000000000000000 ) ) ;
#68976=AXIS2_PLACEMENT_3D ( 'NONE', #80933, #120846, #21351 ) ;
#68977=VECTOR ( 'NONE', #90624, 1000.000000000000000 ) ;
#68978=ORIENTED_EDGE ( 'NONE', *, *, #74426, .F. ) ;
#68979=DIRECTION ( 'NONE',  ( -0.000000000000000000, 1.000000000000000000, -0.000000000000000000 ) ) ;
#68980=CARTESIAN_POINT ( 'NONE',  ( -15.39999999999997904, 2.500000000000000000, 0.000000000000000000 ) ) ;
#68981=EDGE_LOOP ( 'NONE', ( #70489, #102427, #23689, #3722 ) ) ;
#68982=DIRECTION ( 'NONE',  ( 0.000000000000000000, 0.000000000000000000, -1.000000000000000000 ) ) ;
#68983=DIRECTION ( 'NONE',  ( -4.274815082592931898E-19, -0.9999939076577903929, -0.003490651415223739937 ) ) ;
#68984=EDGE_LOOP ( 'NONE', ( #7399, #54195, #87544, #67060 ) ) ;
#68985=VECTOR ( 'NONE', #87820, 1000.000000000000000 ) ;
#68986=CIRCLE ( 'NONE', #18802, 0.06509327318403745899 ) ;
#68987=DIRECTION ( 'NONE',  ( 0.000000000000000000, -0.9999939076577903929, 0.003490651415223739937 ) ) ;
#68988=EDGE_LOOP ( 'NONE', ( #53440, #80710, #35454, #85758 ) ) ;
#68989=ORIENTED_EDGE ( 'NONE', *, *, #74976, .T. ) ;
#68990=LINE ( 'NONE', #78839, #37203 ) ;
#68991=CARTESIAN_POINT ( 'NONE',  ( 7.699999999999925571, 2.500000000000000000, 3.983716857408420076 ) ) ;
#68992=CARTESIAN_POINT ( 'NONE',  ( 1.699999999999951994, 2.500000000000000000, -0.1000000000000022815 ) ) ;
#68993=DIRECTION ( 'NONE',  ( -4.274815082592931898E-19, -0.9999939076577903929, -0.003490651415223739937 ) ) ;
#68995=EDGE_CURVE ( 'NONE', #3294, #18103, #70356, .T. ) ;
#68996=EDGE_LOOP ( 'NONE', ( #127458, #19144, #9971, #41631 ) ) ;
#68997=DIRECTION ( 'NONE',  ( 0.000000000000000000, 0.000000000000000000, -1.000000000000000000 ) ) ;
#68998=ORIENTED_EDGE ( 'NONE', *, *, #91826, .T. ) ;
#68999=CARTESIAN_POINT ( 'NONE',  ( -7.300000000000018474, 12.50000000000000000, 0.4115034346978109769 ) ) ;
#69000=CARTESIAN_POINT ( 'NONE',  ( 11.04999999999991189, 2.500000000000000000, 6.248780366869521430 ) ) ;
#69001=CIRCLE ( 'NONE', #83682, 0.09999999999999999167 ) ;
#69002=ORIENTED_EDGE ( 'NONE', *, *, #90174, .T. ) ;
#69003=DIRECTION ( 'NONE',  ( -0.000000000000000000, -1.000000000000000000, -0.000000000000000000 ) ) ;
#69004=CARTESIAN_POINT ( 'NONE',  ( -10.40000000000000213, 2.500000000000000000, 3.637306695894644726 ) ) ;
#69005=CARTESIAN_POINT ( 'NONE',  ( -8.100000000000010303, 2.500000000000000000, 3.883716857408421319 ) ) ;
#69006=CARTESIAN_POINT ( 'NONE',  ( -7.050000000000016698, 12.50000000000000000, -2.165063509461101710 ) ) ;
#69007=DIRECTION ( 'NONE',  ( 0.000000000000000000, 1.000000000000000000, 0.000000000000000000 ) ) ;
#69008=VERTEX_POINT ( 'NONE', #9280 ) ;
#69009=AXIS2_PLACEMENT_3D ( 'NONE', #111860, #71272, #22203 ) ;
#69010=CARTESIAN_POINT ( 'NONE',  ( 5.849999999999932143, 12.50000000000000000, 2.165063509461097713 ) ) ;
#69011=DIRECTION ( 'NONE',  ( 0.000000000000000000, -0.000000000000000000, 1.000000000000000000 ) ) ;
#69012=DIRECTION ( 'NONE',  ( 0.000000000000000000, 1.000000000000000000, 0.000000000000000000 ) ) ;
#69013=CONICAL_SURFACE ( 'NONE', #71085, 0.09999999999999982514, 0.003490658503988666988 ) ;
#69014=ORIENTED_EDGE ( 'NONE', *, *, #739, .F. ) ;
#69015=CARTESIAN_POINT ( 'NONE',  ( 11.04999999999991189, 2.500000000000000000, 6.148780366869520897 ) ) ;
#69016=AXIS2_PLACEMENT_3D ( 'NONE', #45204, #85109, #35380 ) ;
#69017=AXIS2_PLACEMENT_3D ( 'NONE', #49255, #12368, #109445 ) ;
#69018=VERTEX_POINT ( 'NONE', #28933 ) ;
#69019=ORIENTED_EDGE ( 'NONE', *, *, #125890, .F. ) ;
#69020=DIRECTION ( 'NONE',  ( -0.000000000000000000, 1.000000000000000000, -0.000000000000000000 ) ) ;
#69021=EDGE_LOOP ( 'NONE', ( #67706, #15746, #98547, #43164 ) ) ;
#69022=FACE_OUTER_BOUND ( 'NONE', #74100, .T. ) ;
#69023=DIRECTION ( 'NONE',  ( 0.000000000000000000, 0.000000000000000000, 1.000000000000000000 ) ) ;
#69024=AXIS2_PLACEMENT_3D ( 'NONE', #30105, #70648, #68709 ) ;
#69025=VERTEX_POINT ( 'NONE', #129079 ) ;
#69026=EDGE_CURVE ( 'NONE', #70467, #23771, #39411, .T. ) ;
#69027=FACE_OUTER_BOUND ( 'NONE', #34474, .T. ) ;
#69028=CARTESIAN_POINT ( 'NONE',  ( -12.09999999999999609, 2.500000000000000000, 1.734723475976807094E-15 ) ) ;
#69029=ORIENTED_EDGE ( 'NONE', *, *, #127009, .F. ) ;
#69030=CONICAL_SURFACE ( 'NONE', #117040, 0.1000000000000000056, 0.003490658503988666988 ) ;
#69031=DIRECTION ( 'NONE',  ( 0.000000000000000000, 1.000000000000000000, 0.000000000000000000 ) ) ;
#69032=ADVANCED_FACE ( 'NONE', ( #29560 ), #7647, .T. ) ;
#69033=CARTESIAN_POINT ( 'NONE',  ( -3.750000000000027534, 2.500000000000000000, 2.757883832488649656 ) ) ;
#69034=EDGE_CURVE ( 'NONE', #74274, #124700, #40036, .T. ) ;
#69035=EDGE_LOOP ( 'NONE', ( #12297, #13917 ) ) ;
#69036=ORIENTED_EDGE ( 'NONE', *, *, #72941, .F. ) ;
#69037=ORIENTED_EDGE ( 'NONE', *, *, #89742, .T. ) ;
#69038=CARTESIAN_POINT ( 'NONE',  ( -0.2000000000000339284, 2.500000000000000000, -0.2464101615137759549 ) ) ;
#69039=CARTESIAN_POINT ( 'NONE',  ( 2.899999999999946620, 2.500000000000000000, -3.737306695894649700 ) ) ;
#69040=EDGE_CURVE ( 'NONE', #82957, #79548, #24392, .T. ) ;
#69041=ADVANCED_FACE ( 'NONE', ( #113270 ), #97536, .T. ) ;
#69042=LINE ( 'NONE', #17349, #29597 ) ;
#69043=EDGE_CURVE ( 'NONE', #24381, #64833, #65998, .T. ) ;
#69044=FACE_BOUND ( 'NONE', #62617, .T. ) ;
#69045=ORIENTED_EDGE ( 'NONE', *, *, #32754, .F. ) ;
#69046=EDGE_CURVE ( 'NONE', #16687, #108686, #128969, .T. ) ;
#69047=EDGE_CURVE ( 'NONE', #52849, #81743, #32158, .T. ) ;
#69049=DIRECTION ( 'NONE',  ( 0.000000000000000000, 0.000000000000000000, 1.000000000000000000 ) ) ;
#69050=EDGE_LOOP ( 'NONE', ( #48327, #46387 ) ) ;
#69051=CARTESIAN_POINT ( 'NONE',  ( 7.099999999999927702, 2.500000000000000000, -3.537306695894649966 ) ) ;
#69052=CARTESIAN_POINT ( 'NONE',  ( 17.34779069867720480, 2.317761454549635669, 4.873653559263563473 ) ) ;
#69053=CIRCLE ( 'NONE', #23099, 0.09999999999999982514 ) ;
#69054=CARTESIAN_POINT ( 'NONE',  ( 2.049999999999950084, 2.500000000000000000, 2.065063509461097624 ) ) ;
#69055=DIRECTION ( 'NONE',  ( 0.000000000000000000, 0.000000000000000000, 1.000000000000000000 ) ) ;
#69056=CARTESIAN_POINT ( 'NONE',  ( 0.3999999999999628852, 12.50000000000000000, -0.6277270498435145729 ) ) ;
#69057=VECTOR ( 'NONE', #24053, 1000.000000000000000 ) ;
#69058=ADVANCED_FACE ( 'NONE', ( #72080 ), #83184, .T. ) ;
#69059=CARTESIAN_POINT ( 'NONE',  ( 2.699999999999945555, 12.50000000000000000, 3.983716857408420076 ) ) ;
#69060=CARTESIAN_POINT ( 'NONE',  ( 5.599999999999933031, 2.500000000000000000, -0.3464101615137783474 ) ) ;
#69061=CONICAL_SURFACE ( 'NONE', #33581, 0.1000000000000002554, 0.003490658503988666988 ) ;
#69062=CIRCLE ( 'NONE', #43948, 0.06509327318403745899 ) ;
#69063=VERTEX_POINT ( 'NONE', #14415 ) ;
#69064=ORIENTED_EDGE ( 'NONE', *, *, #23201, .F. ) ;
#69065=ORIENTED_EDGE ( 'NONE', *, *, #78260, .F. ) ;
#69066=EDGE_LOOP ( 'NONE', ( #35600, #106891, #8295, #74311 ) ) ;
#69067=ORIENTED_EDGE ( 'NONE', *, *, #83136, .T. ) ;
#69068=DIRECTION ( 'NONE',  ( -0.000000000000000000, 1.000000000000000000, -0.000000000000000000 ) ) ;
#69069=DIRECTION ( 'NONE',  ( 0.000000000000000000, 0.000000000000000000, 1.000000000000000000 ) ) ;
#69070=ORIENTED_EDGE ( 'NONE', *, *, #128490, .F. ) ;
#69071=FACE_BOUND ( 'NONE', #59341, .T. ) ;
#69072=DIRECTION ( 'NONE',  ( 0.000000000000000000, -0.9999939076577903929, 0.003490651415223739937 ) ) ;
#69073=DIRECTION ( 'NONE',  ( -0.000000000000000000, -1.000000000000000000, -0.000000000000000000 ) ) ;
#69074=CARTESIAN_POINT ( 'NONE',  ( 13.34999999999989662, 12.50000000000000000, -2.230156782645139391 ) ) ;
#69075=DIRECTION ( 'NONE',  ( 0.000000000000000000, 1.000000000000000000, 0.000000000000000000 ) ) ;
#69076=DIRECTION ( 'NONE',  ( 0.000000000000000000, 1.000000000000000000, 0.000000000000000000 ) ) ;
#69077=DIRECTION ( 'NONE',  ( 0.000000000000000000, 0.000000000000000000, 1.000000000000000000 ) ) ;
#69078=ORIENTED_EDGE ( 'NONE', *, *, #58600, .T. ) ;
#69079=ORIENTED_EDGE ( 'NONE', *, *, #120909, .T. ) ;
#69080=VERTEX_POINT ( 'NONE', #43906 ) ;
#69081=ORIENTED_EDGE ( 'NONE', *, *, #34631, .T. ) ;
#69082=EDGE_CURVE ( 'NONE', #40465, #49054, #32816, .T. ) ;
#69083=CARTESIAN_POINT ( 'NONE',  ( 10.79999999999991367, 12.50000000000000000, -2.385244779468109755E-15 ) ) ;
#69084=DIRECTION ( 'NONE',  ( 0.000000000000000000, 0.000000000000000000, 1.000000000000000000 ) ) ;
#69085=ADVANCED_FACE ( 'NONE', ( #53707 ), #51592, .T. ) ;
#69086=VERTEX_POINT ( 'NONE', #72710 ) ;
#69087=DIRECTION ( 'NONE',  ( 0.000000000000000000, 0.000000000000000000, 1.000000000000000000 ) ) ;
#69088=ADVANCED_FACE ( 'NONE', ( #24254 ), #76621, .T. ) ;
#69089=AXIS2_PLACEMENT_3D ( 'NONE', #52409, #112631, #22959 ) ;
#69090=CARTESIAN_POINT ( 'NONE',  ( -0.6500000000000403233, 12.50000000000000000, 1.753560074763284016 ) ) ;
#69091=AXIS2_PLACEMENT_3D ( 'NONE', #77653, #105835, #75721 ) ;
#69092=EDGE_CURVE ( 'NONE', #39004, #23927, #33445, .T. ) ;
#69093=FACE_OUTER_BOUND ( 'NONE', #49412, .T. ) ;
#69095=CARTESIAN_POINT ( 'NONE',  ( -11.24999999999996270, 2.500000000000000000, 2.165063509461097713 ) ) ;
#69097=CARTESIAN_POINT ( 'NONE',  ( -8.150000000000012790, 12.50000000000000000, -2.511473670974877948 ) ) ;
#69098=EDGE_CURVE ( 'NONE', #36428, #118039, #124730, .T. ) ;
#69099=ORIENTED_EDGE ( 'NONE', *, *, #6977, .F. ) ;
#69100=CARTESIAN_POINT ( 'NONE',  ( 8.099999999999921485, 2.500000000000000000, -0.4464101615137783252 ) ) ;
#69101=CIRCLE ( 'NONE', #85819, 0.06509327318403745899 ) ;
#69102=ADVANCED_FACE ( 'NONE', ( #54351 ), #9722, .T. ) ;
#69103=ADVANCED_FACE ( 'NONE', ( #24895 ), #64091, .T. ) ;
#69104=ORIENTED_EDGE ( 'NONE', *, *, #28583, .T. ) ;
#69105=EDGE_CURVE ( 'NONE', #93656, #47134, #85013, .T. ) ;
#69106=ORIENTED_EDGE ( 'NONE', *, *, #33421, .T. ) ;
#69107=CARTESIAN_POINT ( 'NONE',  ( -8.950000000000011724, 12.50000000000000000, -6.148780366869520897 ) ) ;
#69108=FACE_OUTER_BOUND ( 'NONE', #62227, .T. ) ;
#69109=DIRECTION ( 'NONE',  ( 0.000000000000000000, 0.000000000000000000, 1.000000000000000000 ) ) ;
#69110=ORIENTED_EDGE ( 'NONE', *, *, #2874, .T. ) ;
#69111=EDGE_CURVE ( 'NONE', #58857, #43682, #110072, .T. ) ;
#69112=VERTEX_POINT ( 'NONE', #42624 ) ;
#69113=CIRCLE ( 'NONE', #12581, 0.06509327318403745899 ) ;
#69114=DIRECTION ( 'NONE',  ( 0.000000000000000000, 0.000000000000000000, 1.000000000000000000 ) ) ;
#69115=AXIS2_PLACEMENT_3D ( 'NONE', #113803, #44410, #24134 ) ;
#69118=ORIENTED_EDGE ( 'NONE', *, *, #86632, .T. ) ;
#69119=CARTESIAN_POINT ( 'NONE',  ( 6.649999999999930189, 2.500000000000000000, -1.372243186433550033 ) ) ;
#69120=CIRCLE ( 'NONE', #64995, 0.06509327318403745899 ) ;
#69121=ORIENTED_EDGE ( 'NONE', *, *, #125363, .T. ) ;
#69122=CARTESIAN_POINT ( 'NONE',  ( 0.5999999999999555689, 12.50000000000000000, 4.611443907251934426 ) ) ;
#69123=ORIENTED_EDGE ( 'NONE', *, *, #108410, .T. ) ;
#69124=CARTESIAN_POINT ( 'NONE',  ( -3.749999999999991118, 2.500000000000000000, 2.165063509461097713 ) ) ;
#69125=CARTESIAN_POINT ( 'NONE',  ( 1.649999999999951950, 2.500000000000000000, -5.802370205355749988 ) ) ;
#69126=CONICAL_SURFACE ( 'NONE', #123409, 0.1000000000000002554, 0.003490658503988666988 ) ;
#69127=DIRECTION ( 'NONE',  ( 0.000000000000000000, -0.9999939076577903929, 0.003490651415223739937 ) ) ;
#69128=EDGE_CURVE ( 'NONE', #126487, #70798, #13909, .T. ) ;
#69129=DIRECTION ( 'NONE',  ( -0.000000000000000000, -1.000000000000000000, -0.000000000000000000 ) ) ;
#69130=ORIENTED_EDGE ( 'NONE', *, *, #117673, .F. ) ;
#69131=DIRECTION ( 'NONE',  ( -0.000000000000000000, -1.000000000000000000, -0.000000000000000000 ) ) ;
#69133=VERTEX_POINT ( 'NONE', #62891 ) ;
#69134=CARTESIAN_POINT ( 'NONE',  ( -10.85000000000000142, 2.500000000000000000, -2.957883832488649833 ) ) ;
#69135=CARTESIAN_POINT ( 'NONE',  ( 7.049999999999928768, 2.500000000000000000, -2.265063509461101798 ) ) ;
#69136=DIRECTION ( 'NONE',  ( -4.274815082592931898E-19, -0.9999939076577903929, -0.003490651415223739937 ) ) ;
#69137=CARTESIAN_POINT ( 'NONE',  ( -2.300000000000033573, 12.50000000000000000, 0.3464101615137735735 ) ) ;
#69138=DIRECTION ( 'NONE',  ( 0.000000000000000000, 0.000000000000000000, -1.000000000000000000 ) ) ;
#69139=DIRECTION ( 'NONE',  ( 0.000000000000000000, 0.000000000000000000, -1.000000000000000000 ) ) ;
#69140=CARTESIAN_POINT ( 'NONE',  ( 12.49999999999990408, 2.500000000000000000, 5.022947341949748790 ) ) ;
#69141=EDGE_CURVE ( 'NONE', #125929, #18925, #87069, .T. ) ;
#69142=PLANE ( 'NONE',  #32377 ) ;
#69143=DIRECTION ( 'NONE',  ( 0.000000000000000000, 0.000000000000000000, 1.000000000000000000 ) ) ;
#69144=CIRCLE ( 'NONE', #62898, 0.09999999999999982514 ) ;
#69145=AXIS2_PLACEMENT_3D ( 'NONE', #33583, #94409, #4727 ) ;
#69147=ORIENTED_EDGE ( 'NONE', *, *, #70427, .F. ) ;
#69149=CIRCLE ( 'NONE', #37857, 0.06509327318403745899 ) ;
#69150=ADVANCED_FACE ( 'NONE', ( #45195 ), #1487, .T. ) ;
#69151=DIRECTION ( 'NONE',  ( 0.000000000000000000, -0.000000000000000000, 1.000000000000000000 ) ) ;
#69152=CARTESIAN_POINT ( 'NONE',  ( 6.249999999999967137, 2.500000000000000000, -2.165063509461101710 ) ) ;
#69153=CARTESIAN_POINT ( 'NONE',  ( -11.64999999999999680, 12.50000000000000000, -2.165063509461097713 ) ) ;
#69154=DIRECTION ( 'NONE',  ( 0.000000000000000000, 0.000000000000000000, -1.000000000000000000 ) ) ;
#69155=EDGE_LOOP ( 'NONE', ( #121023, #126840, #21228, #44612 ) ) ;
#69156=CARTESIAN_POINT ( 'NONE',  ( -3.750000000000027534, 12.50000000000000000, -1.472243186433550122 ) ) ;
#69157=PLANE ( 'NONE',  #97176 ) ;
#69158=DIRECTION ( 'NONE',  ( 0.000000000000000000, -0.9999939076577903929, 0.003490651415223739937 ) ) ;
#69159=ORIENTED_EDGE ( 'NONE', *, *, #29001, .F. ) ;
#69160=VERTEX_POINT ( 'NONE', #9601 ) ;
#69161=LINE ( 'NONE', #36019, #92752 ) ;
#69162=AXIS2_PLACEMENT_3D ( 'NONE', #76517, #46390, #108548 ) ;
#69163=ORIENTED_EDGE ( 'NONE', *, *, #97919, .F. ) ;
#69164=ORIENTED_EDGE ( 'NONE', *, *, #18496, .T. ) ;
#69165=EDGE_LOOP ( 'NONE', ( #59131, #122514, #2943, #117248 ) ) ;
#69166=PLANE ( 'NONE',  #65397 ) ;
#69167=CARTESIAN_POINT ( 'NONE',  ( 6.449999999999930012, 12.50000000000000000, 6.841600689897072485 ) ) ;
#69168=CARTESIAN_POINT ( 'NONE',  ( 8.349999999999923261, 2.500000000000000000, -6.595190528383302109 ) ) ;
#69169=DIRECTION ( 'NONE',  ( -0.000000000000000000, -1.000000000000000000, -0.000000000000000000 ) ) ;
#69170=AXIS2_PLACEMENT_3D ( 'NONE', #34734, #84456, #26183 ) ;
#69171=ORIENTED_EDGE ( 'NONE', *, *, #89470, .T. ) ;
#69172=CONICAL_SURFACE ( 'NONE', #12738, 0.1000000000000000472, 0.003490658503988666988 ) ;
#69173=EDGE_CURVE ( 'NONE', #103444, #39915, #118559, .T. ) ;
#69174=CARTESIAN_POINT ( 'NONE',  ( -5.400000000000019895, 12.50000000000000000, -0.06509327318403970719 ) ) ;
#69175=ORIENTED_EDGE ( 'NONE', *, *, #106022, .F. ) ;
#69176=CARTESIAN_POINT ( 'NONE',  ( -7.100000000000017408, 12.50000000000000000, -0.6928203230275542523 ) ) ;
#69177=FACE_OUTER_BOUND ( 'NONE', #78482, .T. ) ;
#69178=DIRECTION ( 'NONE',  ( 0.000000000000000000, 0.000000000000000000, 1.000000000000000000 ) ) ;
#69179=DIRECTION ( 'NONE',  ( -0.000000000000000000, 1.000000000000000000, -0.000000000000000000 ) ) ;
#69180=AXIS2_PLACEMENT_3D ( 'NONE', #106688, #57608, #36026 ) ;
#69181=ORIENTED_EDGE ( 'NONE', *, *, #85327, .T. ) ;
#69182=EDGE_LOOP ( 'NONE', ( #75568, #36748, #58863, #118588 ) ) ;
#69183=ORIENTED_EDGE ( 'NONE', *, *, #105921, .T. ) ;
#69184=ORIENTED_EDGE ( 'NONE', *, *, #34808, .T. ) ;
#69185=VERTEX_POINT ( 'NONE', #88128 ) ;
#69186=CARTESIAN_POINT ( 'NONE',  ( 6.449999999999933564, 2.500000000000000000, -6.841600689897078702 ) ) ;
#69187=DIRECTION ( 'NONE',  ( 0.000000000000000000, 0.000000000000000000, 1.000000000000000000 ) ) ;
#69188=EDGE_CURVE ( 'NONE', #39393, #96489, #7737, .T. ) ;
#69189=ADVANCED_FACE ( 'NONE', ( #49543 ), #8299, .T. ) ;
#69190=CARTESIAN_POINT ( 'NONE',  ( 0.5999999999999551248, 2.500000000000000000, -4.576537180435978236 ) ) ;
#69191=EDGE_CURVE ( 'NONE', #52455, #104360, #99710, .T. ) ;
#69192=FACE_BOUND ( 'NONE', #13388, .T. ) ;
#69193=EDGE_CURVE ( 'NONE', #54491, #72352, #107803, .T. ) ;
#69194=DIRECTION ( 'NONE',  ( -0.000000000000000000, 1.000000000000000000, -0.000000000000000000 ) ) ;
#69195=CARTESIAN_POINT ( 'NONE',  ( 0.6499999999999561684, 2.500000000000000000, 1.818653347947321475 ) ) ;
#69196=DIRECTION ( 'NONE',  ( 0.000000000000000000, 0.000000000000000000, 1.000000000000000000 ) ) ;
#69197=DIRECTION ( 'NONE',  ( 0.000000000000000000, 0.000000000000000000, 1.000000000000000000 ) ) ;
#69198=AXIS2_PLACEMENT_3D ( 'NONE', #30737, #97510, #77861 ) ;
#69199=AXIS2_PLACEMENT_3D ( 'NONE', #92716, #73073, #41061 ) ;
#69200=DIRECTION ( 'NONE',  ( -0.000000000000000000, -1.000000000000000000, -0.000000000000000000 ) ) ;
#69201=LINE ( 'NONE', #60700, #105354 ) ;
#69202=EDGE_CURVE ( 'NONE', #2409, #49329, #32917, .T. ) ;
#69203=DIRECTION ( 'NONE',  ( -0.000000000000000000, 1.000000000000000000, -0.000000000000000000 ) ) ;
#69204=AXIS2_PLACEMENT_3D ( 'NONE', #82261, #103179, #90776 ) ;
#69205=ADVANCED_FACE ( 'NONE', ( #38441 ), #18203, .T. ) ;
#69206=EDGE_CURVE ( 'NONE', #123253, #19378, #37005, .T. ) ;
#69208=ORIENTED_EDGE ( 'NONE', *, *, #80704, .T. ) ;
#69209=CIRCLE ( 'NONE', #81733, 0.1000000000000002554 ) ;
#69210=ORIENTED_EDGE ( 'NONE', *, *, #36635, .F. ) ;
#69211=VERTEX_POINT ( 'NONE', #48902 ) ;
#69213=CARTESIAN_POINT ( 'NONE',  ( -11.05000000000000071, 2.500000000000000000, 2.511473670974873507 ) ) ;
#69215=DIRECTION ( 'NONE',  ( 0.000000000000000000, 0.000000000000000000, 1.000000000000000000 ) ) ;
#69216=FACE_BOUND ( 'NONE', #64177, .T. ) ;
#69217=CARTESIAN_POINT ( 'NONE',  ( 9.799999999999918998, 12.50000000000000000, -0.4115034346978156399 ) ) ;
#69218=ORIENTED_EDGE ( 'NONE', *, *, #19227, .F. ) ;
#69219=LINE ( 'NONE', #31898, #4928 ) ;
#69220=DIRECTION ( 'NONE',  ( 0.000000000000000000, 0.000000000000000000, 1.000000000000000000 ) ) ;
#69221=CARTESIAN_POINT ( 'NONE',  ( 7.099999999999928590, 2.500000000000000000, -5.022947341949754119 ) ) ;
#69222=DIRECTION ( 'NONE',  ( 0.000000000000000000, -0.9999939076577903929, 0.003490651415223739937 ) ) ;
#69223=DIRECTION ( 'NONE',  ( 0.000000000000000000, 0.000000000000000000, -1.000000000000000000 ) ) ;
#69225=LINE ( 'NONE', #88881, #40818 ) ;
#69226=ORIENTED_EDGE ( 'NONE', *, *, #59128, .F. ) ;
#69227=AXIS2_PLACEMENT_3D ( 'NONE', #113903, #12459, #112611 ) ;
#69228=EDGE_LOOP ( 'NONE', ( #11876, #46083 ) ) ;
#69229=CIRCLE ( 'NONE', #12793, 0.06509327318403745899 ) ;
#69230=FACE_OUTER_BOUND ( 'NONE', #60610, .T. ) ;
#69231=AXIS2_PLACEMENT_3D ( 'NONE', #84087, #83475, #16627 ) ;
#69232=DIRECTION ( 'NONE',  ( 0.000000000000000000, 1.000000000000000000, 0.000000000000000000 ) ) ;
#69233=EDGE_LOOP ( 'NONE', ( #27323, #95600, #35599, #15330 ) ) ;
#69234=CARTESIAN_POINT ( 'NONE',  ( 0.6499999999999543920, 2.500000000000000000, 6.048780366869521252 ) ) ;
#69235=AXIS2_PLACEMENT_3D ( 'NONE', #597, #18943, #109268 ) ;
#69236=LINE ( 'NONE', #99370, #14364 ) ;
#69237=CONICAL_SURFACE ( 'NONE', #21222, 0.1000000000000000056, 0.003490658503988666988 ) ;
#69238=EDGE_LOOP ( 'NONE', ( #111529, #53813 ) ) ;
#69239=DIRECTION ( 'NONE',  ( 0.000000000000000000, 0.000000000000000000, 1.000000000000000000 ) ) ;
#69241=CARTESIAN_POINT ( 'NONE',  ( -1.050000000000037348, 12.50000000000000000, -6.841600689897078702 ) ) ;
#69242=ORIENTED_EDGE ( 'NONE', *, *, #55509, .T. ) ;
#69243=CARTESIAN_POINT ( 'NONE',  ( -7.500000000000011546, 12.50000000000000000, 3.637306695894644726 ) ) ;
#69244=FACE_BOUND ( 'NONE', #28620, .T. ) ;
#69245=EDGE_CURVE ( 'NONE', #75910, #18522, #106044, .T. ) ;
#69246=ORIENTED_EDGE ( 'NONE', *, *, #5622, .T. ) ;
#69247=CARTESIAN_POINT ( 'NONE',  ( -9.400000000000007461, 12.50000000000000000, -0.3464101615137783474 ) ) ;
#69248=EDGE_CURVE ( 'NONE', #81193, #37867, #55861, .T. ) ;
#69249=ORIENTED_EDGE ( 'NONE', *, *, #99955, .T. ) ;
#69250=DIRECTION ( 'NONE',  ( -4.274815082592931898E-19, -0.9999939076577903929, -0.003490651415223739937 ) ) ;
#69251=DIRECTION ( 'NONE',  ( -4.274815082592931898E-19, -0.9999939076577903929, -0.003490651415223739937 ) ) ;
#69253=DIRECTION ( 'NONE',  ( 0.000000000000000000, -0.9999939076577903929, 0.003490651415223739937 ) ) ;
#69254=DIRECTION ( 'NONE',  ( 0.000000000000000000, -0.9999939076577903929, 0.003490651415223739937 ) ) ;
#69255=ORIENTED_EDGE ( 'NONE', *, *, #36154, .T. ) ;
#69256=EDGE_CURVE ( 'NONE', #91667, #126381, #58071, .T. ) ;
#69257=VERTEX_POINT ( 'NONE', #79009 ) ;
#69258=ORIENTED_EDGE ( 'NONE', *, *, #90524, .T. ) ;
#69259=FACE_OUTER_BOUND ( 'NONE', #108345, .T. ) ;
#69260=CARTESIAN_POINT ( 'NONE',  ( 2.699999999999945555, 2.500000000000000000, 3.983716857408420076 ) ) ;
#69262=ORIENTED_EDGE ( 'NONE', *, *, #101009, .F. ) ;
#69263=VERTEX_POINT ( 'NONE', #5245 ) ;
#69264=ORIENTED_EDGE ( 'NONE', *, *, #93890, .T. ) ;
#69265=FACE_OUTER_BOUND ( 'NONE', #71557, .T. ) ;
#69266=AXIS2_PLACEMENT_3D ( 'NONE', #11687, #51629, #1860 ) ;
#69268=AXIS2_PLACEMENT_3D ( 'NONE', #67023, #16633, #27755 ) ;
#69270=PLANE ( 'NONE',  #15588 ) ;
#69271=CARTESIAN_POINT ( 'NONE',  ( -13.09999999999999254, 12.50000000000000000, 0.3464101615137777923 ) ) ;
#69272=DIRECTION ( 'NONE',  ( 0.000000000000000000, 1.000000000000000000, 0.000000000000000000 ) ) ;
#69273=LINE ( 'NONE', #116445, #49244 ) ;
#69274=DIRECTION ( 'NONE',  ( -0.000000000000000000, 1.000000000000000000, -0.000000000000000000 ) ) ;
#69275=DIRECTION ( 'NONE',  ( 0.000000000000000000, 0.000000000000000000, 1.000000000000000000 ) ) ;
#69276=ORIENTED_EDGE ( 'NONE', *, *, #90354, .F. ) ;
#69277=EDGE_LOOP ( 'NONE', ( #58178, #103642, #34880, #116829 ) ) ;
#69278=CARTESIAN_POINT ( 'NONE',  ( -10.00000000000000533, 2.500000000000000000, 0.5928203230275495006 ) ) ;
#69279=DIRECTION ( 'NONE',  ( 0.000000000000000000, -0.000000000000000000, 1.000000000000000000 ) ) ;
#69280=ORIENTED_EDGE ( 'NONE', *, *, #116555, .F. ) ;
#69282=VERTEX_POINT ( 'NONE', #65452 ) ;
#69284=CARTESIAN_POINT ( 'NONE',  ( 11.64999999999990266, 2.500000000000000000, -6.595190528383302109 ) ) ;
#69285=DIRECTION ( 'NONE',  ( 0.000000000000000000, 0.000000000000000000, 1.000000000000000000 ) ) ;
#69286=CONICAL_SURFACE ( 'NONE', #246, 0.09999999999999982514, 0.003490658503988666988 ) ;
#69287=CARTESIAN_POINT ( 'NONE',  ( -4.600000000000025402, 12.50000000000000000, 0.06509327318403504425 ) ) ;
#69289=CIRCLE ( 'NONE', #100596, 0.06509327318403745899 ) ;
#69292=CARTESIAN_POINT ( 'NONE',  ( -13.14999999999999147, 12.50000000000000000, 1.818653347947325472 ) ) ;
#69293=CIRCLE ( 'NONE', #77610, 0.06509327318403745899 ) ;
#69294=CARTESIAN_POINT ( 'NONE',  ( 2.049999999999950084, 2.500000000000000000, 2.165063509461097713 ) ) ;
#69296=DIRECTION ( 'NONE',  ( 0.000000000000000000, 0.000000000000000000, 1.000000000000000000 ) ) ;
#69297=ORIENTED_EDGE ( 'NONE', *, *, #23426, .F. ) ;
#69298=CIRCLE ( 'NONE', #106957, 0.1000000000000002554 ) ;
#69299=CONICAL_SURFACE ( 'NONE', #56766, 0.1000000000000002554, 0.003490658503988666988 ) ;
#69300=ORIENTED_EDGE ( 'NONE', *, *, #42508, .T. ) ;
#69301=EDGE_CURVE ( 'NONE', #37406, #72308, #16134, .T. ) ;
#69302=ORIENTED_EDGE ( 'NONE', *, *, #52766, .T. ) ;
#69303=EDGE_CURVE ( 'NONE', #25426, #116569, #29258, .T. ) ;
#69304=ORIENTED_EDGE ( 'NONE', *, *, #34651, .F. ) ;
#69305=CARTESIAN_POINT ( 'NONE',  ( -1.850000000000033840, 12.50000000000000000, 6.841600689897072485 ) ) ;
#69306=DIRECTION ( 'NONE',  ( 0.000000000000000000, 0.000000000000000000, 1.000000000000000000 ) ) ;
#69307=ORIENTED_EDGE ( 'NONE', *, *, #46970, .F. ) ;
#69308=FACE_OUTER_BOUND ( 'NONE', #98312, .T. ) ;
#69309=CARTESIAN_POINT ( 'NONE',  ( 7.699999999999923794, 2.500000000000000000, 4.676537180435972552 ) ) ;
#69310=CARTESIAN_POINT ( 'NONE',  ( -1.050000000000037792, 12.50000000000000000, 6.148780366869520009 ) ) ;
#69311=CARTESIAN_POINT ( 'NONE',  ( 15.39999999999989200, 12.50000000000000000, -0.6277270498435167934 ) ) ;
#69312=EDGE_LOOP ( 'NONE', ( #102826, #104072 ) ) ;
#69313=EDGE_CURVE ( 'NONE', #1853, #51752, #78359, .T. ) ;
#69314=CARTESIAN_POINT ( 'NONE',  ( -0.4000000000000331624, 2.500000000000000000, -0.6928203230275519209 ) ) ;
#69315=DIRECTION ( 'NONE',  ( 0.000000000000000000, -0.9999939076577903929, 0.003490651415223739937 ) ) ;
#69316=VERTEX_POINT ( 'NONE', #47605 ) ;
#69317=VERTEX_POINT ( 'NONE', #87499 ) ;
#69319=CIRCLE ( 'NONE', #14920, 0.1000000000000002554 ) ;
#69320=EDGE_LOOP ( 'NONE', ( #28819, #128673 ) ) ;
#69321=CARTESIAN_POINT ( 'NONE',  ( 2.500000000000002220, -1.500000000000000000, 10.00000000000000178 ) ) ;
#69322=AXIS2_PLACEMENT_3D ( 'NONE', #56102, #37133, #77047 ) ;
#69323=CONICAL_SURFACE ( 'NONE', #79803, 0.1000000000000002554, 0.003490658503988666988 ) ;
#69324=B_SPLINE_CURVE_WITH_KNOTS ( 'NONE', 3,
 ( #110967, #53367, #62547, #1666, #41632, #72998, #91993, #121442, #90707, #80896, #31791, #31161, #120809, #63176, #61252, #2303, #112919, #12768, #23240, #123379 ),
 .UNSPECIFIED., .F., .F.,
 ( 4, 2, 2, 2, 2, 2, 2, 2, 2, 4 ),
 ( 0.000000000000000000, 0.0008832438798941733915, 0.001766487759788346783, 0.002649731639682520283, 0.003532975519576693566, 0.005299463279365040566, 0.007065951039153387132, 0.008832438798941733699, 0.01059892655873008287, 0.01413190207830678294 ),
 .UNSPECIFIED. ) ;
#69326=CARTESIAN_POINT ( 'NONE',  ( -10.65000000000000391, 2.500000000000000000, -2.411473670974874306 ) ) ;
#69327=AXIS2_PLACEMENT_3D ( 'NONE', #30095, #20253, #51021 ) ;
#69328=CONICAL_SURFACE ( 'NONE', #58890, 0.1000000000000000472, 0.003490658503988666988 ) ;
#69329=EDGE_CURVE ( 'NONE', #107678, #515, #108436, .T. ) ;
#69330=CIRCLE ( 'NONE', #21316, 0.06509327318403745899 ) ;
#69331=VERTEX_POINT ( 'NONE', #52740 ) ;
#69332=CARTESIAN_POINT ( 'NONE',  ( 0.7999999999999553024, 2.500000000000000000, -4.230127018922201998 ) ) ;
#69333=CARTESIAN_POINT ( 'NONE',  ( -6.505213034913026604E-15, 2.500000000000000000, 4.330127018922196314 ) ) ;
#69334=VECTOR ( 'NONE', #42816, 1000.000000000000000 ) ;
#69335=CARTESIAN_POINT ( 'NONE',  ( -6.050000000000022027, 12.50000000000000000, -6.148780366869526226 ) ) ;
#69336=DIRECTION ( 'NONE',  ( 0.000000000000000000, 1.000000000000000000, 0.000000000000000000 ) ) ;
#69337=CONICAL_SURFACE ( 'NONE', #88196, 0.1000000000000002554, 0.003490658503988666988 ) ;
#69338=ADVANCED_FACE ( 'NONE', ( #70457 ), #92674, .T. ) ;
#69339=ORIENTED_EDGE ( 'NONE', *, *, #91472, .F. ) ;
#69340=CARTESIAN_POINT ( 'NONE',  ( 1.449999999999951328, 2.500000000000000000, 2.611473670974873151 ) ) ;
#69341=ORIENTED_EDGE ( 'NONE', *, *, #73326, .F. ) ;
#69342=ORIENTED_EDGE ( 'NONE', *, *, #51749, .F. ) ;
#69343=CARTESIAN_POINT ( 'NONE',  ( 4.599999999999940137, 2.500000000000000000, -4.330127018922201643 ) ) ;
#69344=ADVANCED_FACE ( 'NONE', ( #62582 ), #116400, .T. ) ;
#69345=ADVANCED_FACE ( 'NONE', ( #101851 ), #85107, .T. ) ;
#69346=LINE ( 'NONE', #107990, #35597 ) ;
#69348=FACE_BOUND ( 'NONE', #56054, .T. ) ;
#69349=ADVANCED_FACE ( 'NONE', ( #3012 ), #92026, .T. ) ;
#69350=DIRECTION ( 'NONE',  ( 0.000000000000000000, 0.000000000000000000, -1.000000000000000000 ) ) ;
#69351=LINE ( 'NONE', #100741, #21458 ) ;
#69352=CARTESIAN_POINT ( 'NONE',  ( 12.09999999999990550, 2.500000000000000000, -4.330127018922201643 ) ) ;
#69353=EDGE_CURVE ( 'NONE', #80440, #86996, #28691, .T. ) ;
#69354=VERTEX_POINT ( 'NONE', #51472 ) ;
#69355=CARTESIAN_POINT ( 'NONE',  ( -1.250000000000035749, 12.50000000000000000, -2.922977105672691422 ) ) ;
#69356=FACE_OUTER_BOUND ( 'NONE', #73168, .T. ) ;
#69357=ADVANCED_FACE ( 'NONE', ( #109743 ), #100553, .T. ) ;
#69358=DIRECTION ( 'NONE',  ( -0.000000000000000000, -1.000000000000000000, -0.000000000000000000 ) ) ;
#69360=ORIENTED_EDGE ( 'NONE', *, *, #53263, .F. ) ;
#69361=CONICAL_SURFACE ( 'NONE', #113279, 0.1000000000000002554, 0.003490658503988666988 ) ;
#69362=DIRECTION ( 'NONE',  ( 0.000000000000000000, 1.000000000000000000, 0.000000000000000000 ) ) ;
#69363=EDGE_CURVE ( 'NONE', #17965, #7615, #60012, .T. ) ;
#69364=ADVANCED_FACE ( 'NONE', ( #40369 ), #22452, .T. ) ;
#69365=DIRECTION ( 'NONE',  ( -0.000000000000000000, -1.000000000000000000, -0.000000000000000000 ) ) ;
#69366=VERTEX_POINT ( 'NONE', #101210 ) ;
#69367=VERTEX_POINT ( 'NONE', #91380 ) ;
#69368=FACE_OUTER_BOUND ( 'NONE', #117124, .T. ) ;
#69369=EDGE_CURVE ( 'NONE', #96946, #17252, #103902, .T. ) ;
#69370=DIRECTION ( 'NONE',  ( -0.000000000000000000, 1.000000000000000000, -0.000000000000000000 ) ) ;
#69371=FACE_BOUND ( 'NONE', #111791, .T. ) ;
#69372=CONICAL_SURFACE ( 'NONE', #52651, 0.1000000000000000472, 0.003490658503988666988 ) ;
#69373=EDGE_CURVE ( 'NONE', #38962, #36641, #82985, .T. ) ;
#69374=CARTESIAN_POINT ( 'NONE',  ( 12.09999999999990550, 2.500000000000000000, -3.537306695894649966 ) ) ;
#69375=CIRCLE ( 'NONE', #21354, 0.06509327318403745899 ) ;
#69376=CIRCLE ( 'NONE', #90293, 0.1000000000000002554 ) ;
#69377=CIRCLE ( 'NONE', #42298, 0.1000000000000002554 ) ;
#69378=LINE ( 'NONE', #109306, #117577 ) ;
#69380=ORIENTED_EDGE ( 'NONE', *, *, #98470, .T. ) ;
#69381=CARTESIAN_POINT ( 'NONE',  ( -5.450000000000023270, 2.500000000000000000, -6.495190528383302464 ) ) ;
#69383=ORIENTED_EDGE ( 'NONE', *, *, #56164, .F. ) ;
#69384=VECTOR ( 'NONE', #71117, 1000.000000000000000 ) ;
#69385=CARTESIAN_POINT ( 'NONE',  ( 8.149999999999920419, 2.500000000000000000, 6.941600689897073018 ) ) ;
#69386=DIRECTION ( 'NONE',  ( 0.000000000000000000, 1.000000000000000000, 0.000000000000000000 ) ) ;
#69387=AXIS2_PLACEMENT_3D ( 'NONE', #123302, #13333, #73545 ) ;
#69388=AXIS2_PLACEMENT_3D ( 'NONE', #106248, #76794, #55224 ) ;
#69389=AXIS2_PLACEMENT_3D ( 'NONE', #35496, #103592, #34207 ) ;
#69390=AXIS2_PLACEMENT_3D ( 'NONE', #56038, #28531, #47528 ) ;
#69391=CARTESIAN_POINT ( 'NONE',  ( 8.749999999999953815, 12.50000000000000000, -2.230156782645139391 ) ) ;
#69392=CARTESIAN_POINT ( 'NONE',  ( 12.09999999999990195, 2.500000000000000000, 0.09999999999999772959 ) ) ;
#69393=VECTOR ( 'NONE', #123304, 1000.000000000000000 ) ;
#69394=VERTEX_POINT ( 'NONE', #42289 ) ;
#69395=DIRECTION ( 'NONE',  ( -0.000000000000000000, 1.000000000000000000, -0.000000000000000000 ) ) ;
#69396=CARTESIAN_POINT ( 'NONE',  ( -10.65000000000000213, 12.50000000000000000, 6.906693963081109722 ) ) ;
#69397=DIRECTION ( 'NONE',  ( 0.000000000000000000, 1.000000000000000000, 0.000000000000000000 ) ) ;
#69398=VERTEX_POINT ( 'NONE', #90078 ) ;
#69399=ORIENTED_EDGE ( 'NONE', *, *, #128901, .F. ) ;
#69400=CARTESIAN_POINT ( 'NONE',  ( 17.46224679592473805, 2.499999999999843237, 5.244174652589637553 ) ) ;
#69401=ORIENTED_EDGE ( 'NONE', *, *, #22622, .T. ) ;
#69402=CARTESIAN_POINT ( 'NONE',  ( 11.69999999999990870, 2.500000000000000000, -4.230127018922201998 ) ) ;
#69403=CARTESIAN_POINT ( 'NONE',  ( 17.50000000000000000, -2.499999999999999556, 1.333333333333338144 ) ) ;
#69404=EDGE_CURVE ( 'NONE', #84934, #40034, #70452, .T. ) ;
#69405=CARTESIAN_POINT ( 'NONE',  ( -7.950000000000016165, 12.50000000000000000, -6.430097255199259010 ) ) ;
#69406=ORIENTED_EDGE ( 'NONE', *, *, #34902, .F. ) ;
#69407=FACE_OUTER_BOUND ( 'NONE', #40957, .T. ) ;
#69408=ADVANCED_FACE ( 'NONE', ( #120844 ), #93437, .T. ) ;
#69409=DIRECTION ( 'NONE',  ( -0.000000000000000000, 1.000000000000000000, -0.000000000000000000 ) ) ;
#69410=CARTESIAN_POINT ( 'NONE',  ( 8.949999999999915801, 2.500000000000000000, 6.941600689897073018 ) ) ;
#69412=DIRECTION ( 'NONE',  ( 0.000000000000000000, 0.000000000000000000, 1.000000000000000000 ) ) ;
#69413=DIRECTION ( 'NONE',  ( 0.000000000000000000, 0.000000000000000000, -1.000000000000000000 ) ) ;
#69414=ORIENTED_EDGE ( 'NONE', *, *, #20613, .F. ) ;
#69415=ORIENTED_EDGE ( 'NONE', *, *, #2414, .T. ) ;
#69416=CARTESIAN_POINT ( 'NONE',  ( 9.999999999999914735, 2.500000000000000000, 0.5928203230275495006 ) ) ;
#69417=VERTEX_POINT ( 'NONE', #120207 ) ;
#69418=AXIS2_PLACEMENT_3D ( 'NONE', #35739, #76952, #16070 ) ;
#69420=AXIS2_PLACEMENT_3D ( 'NONE', #119811, #30159, #10489 ) ;
#69421=EDGE_LOOP ( 'NONE', ( #19929, #63558, #36350, #22746 ) ) ;
#69422=VERTEX_POINT ( 'NONE', #42964 ) ;
#69423=VERTEX_POINT ( 'NONE', #61288 ) ;
#69424=CARTESIAN_POINT ( 'NONE',  ( 0.6499999999999561684, 12.50000000000000000, -1.818653347947325916 ) ) ;
#69425=DIRECTION ( 'NONE',  ( 0.000000000000000000, 0.000000000000000000, 1.000000000000000000 ) ) ;
#69426=AXIS2_PLACEMENT_3D ( 'NONE', #32371, #92534, #37804 ) ;
#69427=AXIS2_PLACEMENT_3D ( 'NONE', #75271, #115172, #94920 ) ;
#69428=FACE_OUTER_BOUND ( 'NONE', #82003, .T. ) ;
#69429=AXIS2_PLACEMENT_3D ( 'NONE', #1335, #20344, #70090 ) ;
#69431=DIRECTION ( 'NONE',  ( 0.000000000000000000, -0.000000000000000000, 1.000000000000000000 ) ) ;
#69432=CARTESIAN_POINT ( 'NONE',  ( 5.599999999999934808, 2.500000000000000000, -3.883716857408426648 ) ) ;
#69433=CARTESIAN_POINT ( 'NONE',  ( -4.251083420886005162E-14, 12.50000000000000000, -3.702399969078687292 ) ) ;
#69434=CIRCLE ( 'NONE', #79909, 0.1000000000000002554 ) ;
#69436=DIRECTION ( 'NONE',  ( 0.000000000000000000, 0.000000000000000000, 1.000000000000000000 ) ) ;
#69437=AXIS2_PLACEMENT_3D ( 'NONE', #92522, #4128, #74180 ) ;
#69438=DIRECTION ( 'NONE',  ( 0.000000000000000000, 0.000000000000000000, -1.000000000000000000 ) ) ;
#69439=CIRCLE ( 'NONE', #33948, 0.06509327318403745899 ) ;
#69440=VERTEX_POINT ( 'NONE', #82866 ) ;
#69441=ORIENTED_EDGE ( 'NONE', *, *, #78854, .T. ) ;
#69443=VERTEX_POINT ( 'NONE', #50193 ) ;
#69444=ORIENTED_EDGE ( 'NONE', *, *, #43513, .F. ) ;
#69445=DIRECTION ( 'NONE',  ( -0.000000000000000000, 1.000000000000000000, -0.000000000000000000 ) ) ;
#69446=EDGE_CURVE ( 'NONE', #102305, #101973, #64180, .T. ) ;
#69448=DIRECTION ( 'NONE',  ( 0.000000000000000000, 0.000000000000000000, 1.000000000000000000 ) ) ;
#69450=DIRECTION ( 'NONE',  ( 0.000000000000000000, 0.000000000000000000, 1.000000000000000000 ) ) ;
#69451=VERTEX_POINT ( 'NONE', #104422 ) ;
#69452=VECTOR ( 'NONE', #125983, 1000.000000000000000 ) ;
#69453=VERTEX_POINT ( 'NONE', #25204 ) ;
#69454=DIRECTION ( 'NONE',  ( 0.000000000000000000, 1.000000000000000000, 0.000000000000000000 ) ) ;
#69455=ORIENTED_EDGE ( 'NONE', *, *, #98475, .F. ) ;
#69456=CARTESIAN_POINT ( 'NONE',  ( 12.29999999999990301, 12.50000000000000000, -0.4115034346978156399 ) ) ;
#69457=ORIENTED_EDGE ( 'NONE', *, *, #125823, .F. ) ;
#69458=ADVANCED_FACE ( 'NONE', ( #73032 ), #39175, .T. ) ;
#69459=EDGE_CURVE ( 'NONE', #54631, #1406, #44207, .T. ) ;
#69460=EDGE_LOOP ( 'NONE', ( #124158, #108848 ) ) ;
#69461=AXIS2_PLACEMENT_3D ( 'NONE', #96546, #36382, #126015 ) ;
#69462=DIRECTION ( 'NONE',  ( 0.000000000000000000, 1.000000000000000000, 0.000000000000000000 ) ) ;
#69463=CARTESIAN_POINT ( 'NONE',  ( 13.09999999999990195, 2.500000000000000000, 3.983716857408420076 ) ) ;
#69464=CIRCLE ( 'NONE', #13014, 0.06509327318403745899 ) ;
#69465=CIRCLE ( 'NONE', #56928, 0.1000000000000002554 ) ;
#69466=CARTESIAN_POINT ( 'NONE',  ( -5.000000000000022204, 2.500000000000000000, -0.6928203230275541413 ) ) ;
#69467=AXIS2_PLACEMENT_3D ( 'NONE', #21862, #98449, #59866 ) ;
#69468=DIRECTION ( 'NONE',  ( -4.274815082592931898E-19, -0.9999939076577903929, -0.003490651415223739937 ) ) ;
#69469=FACE_OUTER_BOUND ( 'NONE', #79040, .T. ) ;
#69470=ORIENTED_EDGE ( 'NONE', *, *, #5535, .T. ) ;
#69471=CARTESIAN_POINT ( 'NONE',  ( -8.150000000000012790, 12.50000000000000000, 2.576566944158910744 ) ) ;
#69472=CARTESIAN_POINT ( 'NONE',  ( 5.649999999999934630, 2.500000000000000000, -1.818653347947325916 ) ) ;
#69473=EDGE_CURVE ( 'NONE', #25044, #75922, #1296, .T. ) ;
#69474=LINE ( 'NONE', #49227, #1886 ) ;
#69475=CARTESIAN_POINT ( 'NONE',  ( 8.349999999999923261, 2.500000000000000000, 2.265063509461097357 ) ) ;
#69476=VECTOR ( 'NONE', #48765, 1000.000000000000000 ) ;
#69477=AXIS2_PLACEMENT_3D ( 'NONE', #86590, #38150, #95778 ) ;
#69478=LINE ( 'NONE', #98951, #62677 ) ;
#69480=AXIS2_PLACEMENT_3D ( 'NONE', #64770, #5838, #7782 ) ;
#69481=CIRCLE ( 'NONE', #2565, 0.06509327318403745899 ) ;
#69482=VERTEX_POINT ( 'NONE', #84126 ) ;
#69483=CARTESIAN_POINT ( 'NONE',  ( 8.949999999999919353, 2.500000000000000000, -6.048780366869526581 ) ) ;
#69484=VECTOR ( 'NONE', #60075, 1000.000000000000000 ) ;
#69485=ORIENTED_EDGE ( 'NONE', *, *, #103913, .T. ) ;
#69486=DIRECTION ( 'NONE',  ( 0.000000000000000000, 0.000000000000000000, 1.000000000000000000 ) ) ;
#69487=CARTESIAN_POINT ( 'NONE',  ( -0.4000000000000392131, 2.500000000000000000, -4.922947341949753586 ) ) ;
#69488=VECTOR ( 'NONE', #52987, 1000.000000000000000 ) ;
#69489=VERTEX_POINT ( 'NONE', #25869 ) ;
#69490=DIRECTION ( 'NONE',  ( -0.000000000000000000, 1.000000000000000000, -0.000000000000000000 ) ) ;
#69491=CARTESIAN_POINT ( 'NONE',  ( -8.350000000000012079, 12.50000000000000000, -2.922977105672691422 ) ) ;
#69492=DIRECTION ( 'NONE',  ( 0.000000000000000000, 0.000000000000000000, 1.000000000000000000 ) ) ;
#69493=DIRECTION ( 'NONE',  ( -0.000000000000000000, -1.000000000000000000, -0.000000000000000000 ) ) ;
#69494=EDGE_CURVE ( 'NONE', #49326, #114386, #33751, .T. ) ;
#69496=ORIENTED_EDGE ( 'NONE', *, *, #98325, .T. ) ;
#69497=EDGE_CURVE ( 'NONE', #97694, #126487, #73662, .T. ) ;
#69498=FACE_OUTER_BOUND ( 'NONE', #104288, .T. ) ;
#69499=CARTESIAN_POINT ( 'NONE',  ( 6.249999999999968914, 2.500000000000000000, -6.495190528383302464 ) ) ;
#69500=EDGE_CURVE ( 'NONE', #43682, #58857, #97722, .T. ) ;
#69501=DIRECTION ( 'NONE',  ( -0.000000000000000000, -1.000000000000000000, -0.000000000000000000 ) ) ;
#69502=ORIENTED_EDGE ( 'NONE', *, *, #60903, .T. ) ;
#69503=DIRECTION ( 'NONE',  ( 0.000000000000000000, 0.000000000000000000, 1.000000000000000000 ) ) ;
#69504=VECTOR ( 'NONE', #86100, 1000.000000000000000 ) ;
#69505=AXIS2_PLACEMENT_3D ( 'NONE', #42562, #62200, #32742 ) ;
#69506=EDGE_CURVE ( 'NONE', #67824, #83209, #14087, .T. ) ;
#69507=CIRCLE ( 'NONE', #54839, 0.1000000000000000472 ) ;
#69508=ADVANCED_FACE ( 'NONE', ( #35695 ), #115510, .T. ) ;
#69509=VERTEX_POINT ( 'NONE', #55334 ) ;
#69510=CARTESIAN_POINT ( 'NONE',  ( 1.249999999999953815, 12.50000000000000000, 1.537336459617582918 ) ) ;
#69511=PLANE ( 'NONE',  #40421 ) ;
#69512=ADVANCED_FACE ( 'NONE', ( #35061 ), #114446, .T. ) ;
#69513=DIRECTION ( 'NONE',  ( 0.000000000000000000, 0.000000000000000000, 1.000000000000000000 ) ) ;
#69514=VERTEX_POINT ( 'NONE', #33127 ) ;
#69515=CIRCLE ( 'NONE', #117715, 0.1000000000000002554 ) ;
#69516=CARTESIAN_POINT ( 'NONE',  ( 10.39999999999991509, 12.50000000000000000, -0.7579135962115917113 ) ) ;
#69517=AXIS2_PLACEMENT_3D ( 'NONE', #18284, #20231, #108604 ) ;
#69518=CIRCLE ( 'NONE', #54948, 0.1000000000000002554 ) ;
#69519=EDGE_CURVE ( 'NONE', #37534, #54491, #28786, .T. ) ;
#69520=DIRECTION ( 'NONE',  ( -0.000000000000000000, 1.000000000000000000, -0.000000000000000000 ) ) ;
#69521=CIRCLE ( 'NONE', #115481, 0.06509327318403745899 ) ;
#69522=ORIENTED_EDGE ( 'NONE', *, *, #51079, .T. ) ;
#69523=CONICAL_SURFACE ( 'NONE', #123802, 0.1000000000000000472, 0.003490658503988666988 ) ;
#69524=DIRECTION ( 'NONE',  ( 0.000000000000000000, 1.000000000000000000, 0.000000000000000000 ) ) ;
#69525=EDGE_LOOP ( 'NONE', ( #13915, #46869 ) ) ;
#69526=ADVANCED_FACE ( 'NONE', ( #113602 ), #4917, .T. ) ;
#69527=AXIS2_PLACEMENT_3D ( 'NONE', #18757, #49528, #89439 ) ;
#69528=DIRECTION ( 'NONE',  ( 0.000000000000000000, 0.000000000000000000, 1.000000000000000000 ) ) ;
#69529=EDGE_LOOP ( 'NONE', ( #96300, #7007 ) ) ;
#69530=DIRECTION ( 'NONE',  ( 0.000000000000000000, 0.000000000000000000, -1.000000000000000000 ) ) ;
#69531=CARTESIAN_POINT ( 'NONE',  ( 8.328334240990686865, 2.499999999999999556, -8.539519492767928099 ) ) ;
#69532=VERTEX_POINT ( 'NONE', #3645 ) ;
#69533=EDGE_LOOP ( 'NONE', ( #91825, #57368 ) ) ;
#69534=CARTESIAN_POINT ( 'NONE',  ( -7.700000000000014388, 2.500000000000000000, -4.776537180435977525 ) ) ;
#69536=EDGE_LOOP ( 'NONE', ( #80707, #47775, #77006, #11327 ) ) ;
#69537=AXIS2_PLACEMENT_3D ( 'NONE', #116830, #66447, #106375 ) ;
#69538=LINE ( 'NONE', #48624, #119891 ) ;
#69539=CARTESIAN_POINT ( 'NONE',  ( 4.199999999999939782, 12.50000000000000000, -2.276824562219559311E-15 ) ) ;
#69540=DIRECTION ( 'NONE',  ( -0.000000000000000000, -1.000000000000000000, -0.000000000000000000 ) ) ;
#69541=CARTESIAN_POINT ( 'NONE',  ( -3.350000000000028511, 2.500000000000000000, 2.857883832488649301 ) ) ;
#69542=CARTESIAN_POINT ( 'NONE',  ( 7.499999999999925393, 12.50000000000000000, -0.6928203230275541413 ) ) ;
#69543=LINE ( 'NONE', #68255, #95341 ) ;
#69544=DIRECTION ( 'NONE',  ( 0.000000000000000000, 0.000000000000000000, -1.000000000000000000 ) ) ;
#69545=VECTOR ( 'NONE', #72886, 1000.000000000000000 ) ;
#69546=CIRCLE ( 'NONE', #102999, 1.000000000000000888 ) ;
#69547=AXIS2_PLACEMENT_3D ( 'NONE', #111398, #123179, #93081 ) ;
#69548=EDGE_LOOP ( 'NONE', ( #43523, #55662, #37837, #50803 ) ) ;
#69549=ORIENTED_EDGE ( 'NONE', *, *, #58462, .F. ) ;
#69550=ORIENTED_EDGE ( 'NONE', *, *, #1504, .F. ) ;
#69551=ORIENTED_EDGE ( 'NONE', *, *, #52778, .T. ) ;
#69552=CARTESIAN_POINT ( 'NONE',  ( 4.999999999999969802, 12.50000000000000000, 4.330127018922196314 ) ) ;
#69553=DIRECTION ( 'NONE',  ( 0.000000000000000000, 0.000000000000000000, 1.000000000000000000 ) ) ;
#69554=DIRECTION ( 'NONE',  ( 0.000000000000000000, 1.000000000000000000, 0.000000000000000000 ) ) ;
#69555=ORIENTED_EDGE ( 'NONE', *, *, #43572, .F. ) ;
#69556=FACE_BOUND ( 'NONE', #50432, .T. ) ;
#69557=VERTEX_POINT ( 'NONE', #24575 ) ;
#69558=CONICAL_SURFACE ( 'NONE', #90479, 0.1000000000000002554, 0.003490658503988666988 ) ;
#69559=CARTESIAN_POINT ( 'NONE',  ( -10.80000000000000249, 2.500000000000000000, -4.430127018922197735 ) ) ;
#69560=CARTESIAN_POINT ( 'NONE',  ( 5.649999999999936406, 2.500000000000000000, -6.248780366869526759 ) ) ;
#69561=AXIS2_PLACEMENT_3D ( 'NONE', #8428, #128892, #99419 ) ;
#69562=VECTOR ( 'NONE', #116575, 1000.000000000000000 ) ;
#69563=DIRECTION ( 'NONE',  ( 0.000000000000000000, 1.000000000000000000, 0.000000000000000000 ) ) ;
#69564=AXIS2_PLACEMENT_3D ( 'NONE', #57759, #85898, #17135 ) ;
#69565=ADVANCED_FACE ( 'NONE', ( #83513 ), #43594, .T. ) ;
#69566=DIRECTION ( 'NONE',  ( 0.000000000000000000, 0.000000000000000000, 1.000000000000000000 ) ) ;
#69567=CARTESIAN_POINT ( 'NONE',  ( -11.84999999999999609, 2.500000000000000000, 1.918653347947321564 ) ) ;
#69568=CARTESIAN_POINT ( 'NONE',  ( 2.899999999999943956, 12.50000000000000000, 4.265033745738159077 ) ) ;
#69569=DIRECTION ( 'NONE',  ( 0.000000000000000000, 0.000000000000000000, 1.000000000000000000 ) ) ;
#69570=DIRECTION ( 'NONE',  ( 0.000000000000000000, -0.000000000000000000, 1.000000000000000000 ) ) ;
#69571=CARTESIAN_POINT ( 'NONE',  ( 2.099999999999949463, 12.50000000000000000, 0.6928203230275494784 ) ) ;
#69572=DIRECTION ( 'NONE',  ( -0.000000000000000000, -1.000000000000000000, -0.000000000000000000 ) ) ;
#69573=VECTOR ( 'NONE', #18349, 1000.000000000000000 ) ;
#69574=EDGE_CURVE ( 'NONE', #24791, #77492, #54662, .T. ) ;
#69575=ORIENTED_EDGE ( 'NONE', *, *, #30978, .T. ) ;
#69576=ORIENTED_EDGE ( 'NONE', *, *, #101029, .T. ) ;
#69577=EDGE_LOOP ( 'NONE', ( #3038, #106711, #116651, #127010 ) ) ;
#69578=VECTOR ( 'NONE', #77806, 1000.000000000000000 ) ;
#69579=ORIENTED_EDGE ( 'NONE', *, *, #18224, .T. ) ;
#69580=AXIS2_PLACEMENT_3D ( 'NONE', #21994, #12135, #112294 ) ;
#69581=VECTOR ( 'NONE', #83123, 1000.000000000000000 ) ;
#69582=DIRECTION ( 'NONE',  ( 0.000000000000000000, 0.000000000000000000, 1.000000000000000000 ) ) ;
#69583=DIRECTION ( 'NONE',  ( -0.000000000000000000, 1.000000000000000000, -0.000000000000000000 ) ) ;
#69584=ORIENTED_EDGE ( 'NONE', *, *, #21943, .T. ) ;
#69585=ORIENTED_EDGE ( 'NONE', *, *, #115753, .F. ) ;
#69586=ORIENTED_EDGE ( 'NONE', *, *, #121799, .T. ) ;
#69587=AXIS2_PLACEMENT_3D ( 'NONE', #3703, #113667, #63926 ) ;
#69588=DIRECTION ( 'NONE',  ( 0.000000000000000000, 0.000000000000000000, 1.000000000000000000 ) ) ;
#69589=DIRECTION ( 'NONE',  ( 0.000000000000000000, -0.9999939076577903929, 0.003490651415223739937 ) ) ;
#69590=AXIS2_PLACEMENT_3D ( 'NONE', #38525, #47041, #67949 ) ;
#69591=CARTESIAN_POINT ( 'NONE',  ( -2.100000000000033396, 12.50000000000000000, -5.022947341949754119 ) ) ;
#69592=DIRECTION ( 'NONE',  ( 0.000000000000000000, 1.000000000000000000, 0.000000000000000000 ) ) ;
#69593=CARTESIAN_POINT ( 'NONE',  ( 11.69999999999990514, 2.500000000000000000, -2.276824562219559311E-15 ) ) ;
#69595=DIRECTION ( 'NONE',  ( 0.000000000000000000, -0.9999939076577903929, 0.003490651415223739937 ) ) ;
#69596=EDGE_LOOP ( 'NONE', ( #25793, #76914, #124848, #112823 ) ) ;
#69597=DIRECTION ( 'NONE',  ( 0.000000000000000000, 1.000000000000000000, 0.000000000000000000 ) ) ;
#69598=VERTEX_POINT ( 'NONE', #45521 ) ;
#69599=EDGE_LOOP ( 'NONE', ( #75212, #84493 ) ) ;
#69600=ORIENTED_EDGE ( 'NONE', *, *, #63324, .T. ) ;
#69601=FACE_OUTER_BOUND ( 'NONE', #22079, .T. ) ;
#69602=AXIS2_PLACEMENT_3D ( 'NONE', #94236, #54319, #123064 ) ;
#69603=VECTOR ( 'NONE', #98779, 1000.000000000000000 ) ;
#69604=EDGE_LOOP ( 'NONE', ( #88413, #73979, #86052, #26937 ) ) ;
#69605=EDGE_LOOP ( 'NONE', ( #55149, #6581, #117511, #19834 ) ) ;
#69606=DIRECTION ( 'NONE',  ( 0.000000000000000000, -0.9999939076577903929, 0.003490651415223739937 ) ) ;
#69607=EDGE_CURVE ( 'NONE', #78336, #4391, #103784, .T. ) ;
#69608=VECTOR ( 'NONE', #33303, 1000.000000000000000 ) ;
#69609=DIRECTION ( 'NONE',  ( 0.000000000000000000, 0.000000000000000000, 1.000000000000000000 ) ) ;
#69610=DIRECTION ( 'NONE',  ( 0.000000000000000000, 1.000000000000000000, 0.000000000000000000 ) ) ;
#69611=DIRECTION ( 'NONE',  ( 0.000000000000000000, 0.000000000000000000, 1.000000000000000000 ) ) ;
#69612=AXIS2_PLACEMENT_3D ( 'NONE', #33234, #73765, #71194 ) ;
#69613=AXIS2_PLACEMENT_3D ( 'NONE', #5548, #86027, #26501 ) ;
#69615=ORIENTED_EDGE ( 'NONE', *, *, #267, .T. ) ;
#69616=DIRECTION ( 'NONE',  ( 0.000000000000000000, 0.000000000000000000, 1.000000000000000000 ) ) ;
#69617=ADVANCED_FACE ( 'NONE', ( #14096 ), #103719, .T. ) ;
#69618=AXIS2_PLACEMENT_3D ( 'NONE', #78691, #30239, #28289 ) ;
#69619=CONICAL_SURFACE ( 'NONE', #119789, 0.1000000000000000472, 0.003490658503988666988 ) ;
#69620=ORIENTED_EDGE ( 'NONE', *, *, #70036, .F. ) ;
#69621=DIRECTION ( 'NONE',  ( 0.000000000000000000, -0.000000000000000000, 1.000000000000000000 ) ) ;
#69622=AXIS2_PLACEMENT_3D ( 'NONE', #63052, #52582, #91225 ) ;
#69623=VERTEX_POINT ( 'NONE', #8788 ) ;
#69625=DIRECTION ( 'NONE',  ( 0.000000000000000000, -0.000000000000000000, 1.000000000000000000 ) ) ;
#69626=AXIS2_PLACEMENT_3D ( 'NONE', #31300, #83613, #71859 ) ;
#69627=EDGE_LOOP ( 'NONE', ( #4028, #10843 ) ) ;
#69628=DIRECTION ( 'NONE',  ( 0.000000000000000000, 1.000000000000000000, 0.000000000000000000 ) ) ;
#69629=ADVANCED_FACE ( 'NONE', ( #46803 ), #127300, .T. ) ;
#69630=CARTESIAN_POINT ( 'NONE',  ( -0.4500000000000397571, 12.50000000000000000, -6.495190528383302464 ) ) ;
#69631=EDGE_CURVE ( 'NONE', #10759, #32556, #91465, .T. ) ;
#69632=ORIENTED_EDGE ( 'NONE', *, *, #41781, .F. ) ;
#69633=VECTOR ( 'NONE', #12486, 1000.000000000000000 ) ;
#69634=EDGE_CURVE ( 'NONE', #15926, #44661, #108917, .T. ) ;
#69635=LINE ( 'NONE', #12000, #744 ) ;
#69636=EDGE_LOOP ( 'NONE', ( #121150, #45341 ) ) ;
#69637=ORIENTED_EDGE ( 'NONE', *, *, #67725, .F. ) ;
#69638=PLANE ( 'NONE',  #108286 ) ;
#69639=LINE ( 'NONE', #91865, #53458 ) ;
#69640=ADVANCED_FACE ( 'NONE', ( #97820 ), #12041, .T. ) ;
#69641=FACE_OUTER_BOUND ( 'NONE', #108253, .T. ) ;
#69642=DIRECTION ( 'NONE',  ( -0.000000000000000000, 1.000000000000000000, -0.000000000000000000 ) ) ;
#69643=AXIS2_PLACEMENT_3D ( 'NONE', #107518, #36856, #7368 ) ;
#69645=ORIENTED_EDGE ( 'NONE', *, *, #50326, .F. ) ;
#69646=FACE_OUTER_BOUND ( 'NONE', #88104, .T. ) ;
#69647=AXIS2_PLACEMENT_3D ( 'NONE', #1883, #61478, #60819 ) ;
#69648=VERTEX_POINT ( 'NONE', #58562 ) ;
#69649=CONICAL_SURFACE ( 'NONE', #23677, 0.1000000000000000056, 0.003490658503988666988 ) ;
#69650=CARTESIAN_POINT ( 'NONE',  ( 8.149999999999920419, 2.500000000000000000, -2.611473670974877592 ) ) ;
#69651=FACE_OUTER_BOUND ( 'NONE', #1389, .T. ) ;
#69652=CARTESIAN_POINT ( 'NONE',  ( 9.799999999999915445, 2.500000000000000000, -4.676537180435977881 ) ) ;
#69653=FACE_OUTER_BOUND ( 'NONE', #50649, .T. ) ;
#69654=CARTESIAN_POINT ( 'NONE',  ( -1.450000000000035483, 12.50000000000000000, 6.148780366869520897 ) ) ;
#69655=CARTESIAN_POINT ( 'NONE',  ( -6.250000000000021316, 2.500000000000000000, -5.802370205355749988 ) ) ;
#69656=AXIS2_PLACEMENT_3D ( 'NONE', #55541, #35263, #24788 ) ;
#69657=FACE_OUTER_BOUND ( 'NONE', #49476, .T. ) ;
#69658=CIRCLE ( 'NONE', #109370, 0.06509327318403745899 ) ;
#69659=ORIENTED_EDGE ( 'NONE', *, *, #58729, .F. ) ;
#69660=AXIS2_PLACEMENT_3D ( 'NONE', #68449, #16756, #56682 ) ;
#69661=LINE ( 'NONE', #39595, #47996 ) ;
#69662=DIRECTION ( 'NONE',  ( 0.000000000000000000, 0.000000000000000000, -1.000000000000000000 ) ) ;
#69664=ORIENTED_EDGE ( 'NONE', *, *, #74794, .T. ) ;
#69665=EDGE_CURVE ( 'NONE', #76961, #113506, #108179, .T. ) ;
#69666=LINE ( 'NONE', #120706, #113772 ) ;
#69667=EDGE_LOOP ( 'NONE', ( #65143, #42609, #64271, #47168 ) ) ;
#69668=VECTOR ( 'NONE', #122015, 1000.000000000000000 ) ;
#69669=AXIS2_PLACEMENT_3D ( 'NONE', #77513, #27762, #57891 ) ;
#69670=ORIENTED_EDGE ( 'NONE', *, *, #73455, .F. ) ;
#69671=CONICAL_SURFACE ( 'NONE', #40452, 0.1000000000000002554, 0.003490658503988666988 ) ;
#69672=CARTESIAN_POINT ( 'NONE',  ( 6.049999999999934097, 2.500000000000000000, -6.148780366869526226 ) ) ;
#69673=ADVANCED_FACE ( 'NONE', ( #28457 ), #57916, .T. ) ;
#69674=ADVANCED_FACE ( 'NONE', ( #27786 ), #47284, .T. ) ;
#69675=CONICAL_SURFACE ( 'NONE', #65567, 0.09999999999999982514, 0.003490658503988666988 ) ;
#69676=VERTEX_POINT ( 'NONE', #98453 ) ;
#69677=CARTESIAN_POINT ( 'NONE',  ( -0.6500000000000394351, 12.50000000000000000, 2.511473670974873507 ) ) ;
#69678=CARTESIAN_POINT ( 'NONE',  ( -7.100000000000018296, 12.50000000000000000, -4.330127018922201643 ) ) ;
#69679=ADVANCED_FACE ( 'NONE', ( #8146 ), #91187, .T. ) ;
#69680=EDGE_CURVE ( 'NONE', #119313, #58497, #64278, .T. ) ;
#69681=ORIENTED_EDGE ( 'NONE', *, *, #62514, .F. ) ;
#69682=CARTESIAN_POINT ( 'NONE',  ( 4.599999999999936584, 2.500000000000000000, 3.537306695894645081 ) ) ;
#69683=ADVANCED_FACE ( 'NONE', ( #29110 ), #124641, .T. ) ;
#69684=DIRECTION ( 'NONE',  ( 0.000000000000000000, -0.9999939076577903929, 0.003490651415223739937 ) ) ;
#69685=DIRECTION ( 'NONE',  ( 0.000000000000000000, -0.000000000000000000, 1.000000000000000000 ) ) ;
#69686=ORIENTED_EDGE ( 'NONE', *, *, #122929, .F. ) ;
#69687=EDGE_CURVE ( 'NONE', #97846, #22678, #68188, .T. ) ;
#69688=EDGE_CURVE ( 'NONE', #87824, #91861, #57750, .T. ) ;
#69689=EDGE_LOOP ( 'NONE', ( #34451, #43166 ) ) ;
#69690=VERTEX_POINT ( 'NONE', #66427 ) ;
#69691=DIRECTION ( 'NONE',  ( 0.000000000000000000, 1.000000000000000000, 0.000000000000000000 ) ) ;
#69692=FACE_OUTER_BOUND ( 'NONE', #124653, .T. ) ;
#69693=CIRCLE ( 'NONE', #67629, 0.06509327318403745899 ) ;
#69694=CARTESIAN_POINT ( 'NONE',  ( -13.94999999999998685, 2.500000000000000000, -2.511473670974875727 ) ) ;
#69695=AXIS2_PLACEMENT_3D ( 'NONE', #107740, #59309, #19344 ) ;
#69696=FACE_BOUND ( 'NONE', #68333, .T. ) ;
#69697=EDGE_LOOP ( 'NONE', ( #97885, #8128, #45587, #47673 ) ) ;
#69698=DIRECTION ( 'NONE',  ( 0.000000000000000000, 1.000000000000000000, 0.000000000000000000 ) ) ;
#69699=CARTESIAN_POINT ( 'NONE',  ( 1.449999999999949551, 2.500000000000000000, 6.841600689897072485 ) ) ;
#69700=EDGE_LOOP ( 'NONE', ( #80654, #37373, #114111, #65154 ) ) ;
#69701=FACE_OUTER_BOUND ( 'NONE', #74208, .T. ) ;
#69702=AXIS2_PLACEMENT_3D ( 'NONE', #44892, #25884, #14112 ) ;
#69703=CARTESIAN_POINT ( 'NONE',  ( -7.100000000000017408, 2.500000000000000000, -0.5928203230275542746 ) ) ;
#69704=AXIS2_PLACEMENT_3D ( 'NONE', #3792, #95395, #124858 ) ;
#69705=AXIS2_PLACEMENT_3D ( 'NONE', #86936, #8368, #48969 ) ;
#69707=CARTESIAN_POINT ( 'NONE',  ( 87.50000000000002842, 4.028096841260344525E-16, 7.500000000000000888 ) ) ;
#69708=CONICAL_SURFACE ( 'NONE', #44679, 0.1000000000000000472, 0.003490658503988666988 ) ;
#69709=FACE_OUTER_BOUND ( 'NONE', #49662, .T. ) ;
#69710=CARTESIAN_POINT ( 'NONE',  ( -1.900000000000034106, 12.50000000000000000, -3.983716857408426293 ) ) ;
#69711=DIRECTION ( 'NONE',  ( -4.274815082592931898E-19, -0.9999939076577903929, -0.003490651415223739937 ) ) ;
#69712=LINE ( 'NONE', #120743, #123500 ) ;
#69713=CONICAL_SURFACE ( 'NONE', #13264, 0.1000000000000002554, 0.003490658503988666988 ) ;
#69714=VECTOR ( 'NONE', #118689, 1000.000000000000000 ) ;
#69715=CIRCLE ( 'NONE', #115769, 0.06509327318403745899 ) ;
#69716=ORIENTED_EDGE ( 'NONE', *, *, #58854, .T. ) ;
#69717=ORIENTED_EDGE ( 'NONE', *, *, #61301, .T. ) ;
#69718=EDGE_LOOP ( 'NONE', ( #37602, #13678, #89865, #71174 ) ) ;
#69719=ORIENTED_EDGE ( 'NONE', *, *, #91416, .T. ) ;
#69720=CIRCLE ( 'NONE', #52996, 0.09999999999999982514 ) ;
#69721=ORIENTED_EDGE ( 'NONE', *, *, #20665, .F. ) ;
#69722=CARTESIAN_POINT ( 'NONE',  ( -6.249999999999981348, 12.50000000000000000, 6.495190528383297135 ) ) ;
#69723=AXIS2_PLACEMENT_3D ( 'NONE', #125167, #64305, #93139 ) ;
#69724=CARTESIAN_POINT ( 'NONE',  ( 11.24999999999990941, 2.500000000000000000, 7.188010851410848723 ) ) ;
#69725=ORIENTED_EDGE ( 'NONE', *, *, #28757, .T. ) ;
#69726=FACE_BOUND ( 'NONE', #70924, .T. ) ;
#69727=LINE ( 'NONE', #19319, #70857 ) ;
#69728=DIRECTION ( 'NONE',  ( 0.000000000000000000, 0.000000000000000000, 1.000000000000000000 ) ) ;
#69729=CARTESIAN_POINT ( 'NONE',  ( -0.6500000000000394351, 2.500000000000000000, 6.841600689897072485 ) ) ;
#69730=PLANE ( 'NONE',  #30787 ) ;
#69731=DIRECTION ( 'NONE',  ( 0.000000000000000000, -0.000000000000000000, 1.000000000000000000 ) ) ;
#69732=CARTESIAN_POINT ( 'NONE',  ( 1.649999999999951505, 2.500000000000000000, 1.372243186433545370 ) ) ;
#69733=VERTEX_POINT ( 'NONE', #19249 ) ;
#69734=CIRCLE ( 'NONE', #86443, 0.09999999999999982514 ) ;
#69735=VERTEX_POINT ( 'NONE', #59213 ) ;
#69736=ADVANCED_FACE ( 'NONE', ( #108287 ), #93528, .T. ) ;
#69737=ORIENTED_EDGE ( 'NONE', *, *, #66308, .T. ) ;
#69738=ORIENTED_EDGE ( 'NONE', *, *, #73924, .F. ) ;
#69739=ORIENTED_EDGE ( 'NONE', *, *, #7416, .T. ) ;
#69740=DIRECTION ( 'NONE',  ( 0.000000000000000000, 0.000000000000000000, 1.000000000000000000 ) ) ;
#69741=ORIENTED_EDGE ( 'NONE', *, *, #47334, .T. ) ;
#69742=DIRECTION ( 'NONE',  ( 0.000000000000000000, 0.000000000000000000, 1.000000000000000000 ) ) ;
#69743=AXIS2_PLACEMENT_3D ( 'NONE', #14472, #75340, #34804 ) ;
#69744=AXIS2_PLACEMENT_3D ( 'NONE', #71445, #9482, #7532 ) ;
#69745=CARTESIAN_POINT ( 'NONE',  ( -8.750000000000010658, 2.500000000000000000, 2.757883832488649656 ) ) ;
#69746=DIRECTION ( 'NONE',  ( 0.000000000000000000, 1.000000000000000000, 0.000000000000000000 ) ) ;
#69748=DIRECTION ( 'NONE',  ( -0.000000000000000000, -1.000000000000000000, -0.000000000000000000 ) ) ;
#69749=CARTESIAN_POINT ( 'NONE',  ( 8.099999999999923261, 2.500000000000000000, 4.576537180435972019 ) ) ;
#69750=CARTESIAN_POINT ( 'NONE',  ( 2.499999999999948930, 2.500000000000000000, -5.022947341949754119 ) ) ;
#69751=CONICAL_SURFACE ( 'NONE', #61454, 0.1000000000000000056, 0.003490658503988666988 ) ;
#69752=VERTEX_POINT ( 'NONE', #116166 ) ;
#69753=DIRECTION ( 'NONE',  ( 0.000000000000000000, 0.000000000000000000, 1.000000000000000000 ) ) ;
#69754=CONICAL_SURFACE ( 'NONE', #59318, 0.09999999999999982514, 0.003490658503988666988 ) ;
#69755=CONICAL_SURFACE ( 'NONE', #44729, 0.1000000000000002554, 0.003490658503988666988 ) ;
#69756=EDGE_LOOP ( 'NONE', ( #73336, #39987, #13718, #94546 ) ) ;
#69757=AXIS2_PLACEMENT_3D ( 'NONE', #64506, #4274, #15391 ) ;
#69758=EDGE_LOOP ( 'NONE', ( #70383, #101224, #63589, #79096 ) ) ;
#69759=DIRECTION ( 'NONE',  ( 0.000000000000000000, 0.000000000000000000, 1.000000000000000000 ) ) ;
#69760=LINE ( 'NONE', #60607, #53141 ) ;
#69761=LINE ( 'NONE', #19355, #6998 ) ;
#69762=AXIS2_PLACEMENT_3D ( 'NONE', #29191, #58645, #69084 ) ;
#69763=ORIENTED_EDGE ( 'NONE', *, *, #81448, .T. ) ;
#69764=ORIENTED_EDGE ( 'NONE', *, *, #35785, .T. ) ;
#69765=DIRECTION ( 'NONE',  ( 0.000000000000000000, -0.000000000000000000, 1.000000000000000000 ) ) ;
#69766=CARTESIAN_POINT ( 'NONE',  ( 9.149999999999915090, 2.500000000000000000, -2.265063509461101798 ) ) ;
#69767=AXIS2_PLACEMENT_3D ( 'NONE', #24453, #14606, #55210 ) ;
#69768=CARTESIAN_POINT ( 'NONE',  ( 11.84999999999990727, 2.500000000000000000, -2.611473670974877592 ) ) ;
#69769=AXIS2_PLACEMENT_3D ( 'NONE', #109322, #119787, #117833 ) ;
#69770=CONICAL_SURFACE ( 'NONE', #53055, 0.09999999999999982514, 0.003490658503988666988 ) ;
#69771=FACE_OUTER_BOUND ( 'NONE', #43558, .T. ) ;
#69772=VERTEX_POINT ( 'NONE', #26515 ) ;
#69773=PLANE ( 'NONE',  #98296 ) ;
#69774=ORIENTED_EDGE ( 'NONE', *, *, #21140, .F. ) ;
#69775=CARTESIAN_POINT ( 'NONE',  ( 1.699999999999951994, 12.50000000000000000, 0.06509327318403515528 ) ) ;
#69776=ADVANCED_FACE ( 'NONE', ( #56593 ), #36979, .T. ) ;
#69777=ORIENTED_EDGE ( 'NONE', *, *, #25110, .F. ) ;
#69779=CARTESIAN_POINT ( 'NONE',  ( -5.450000000000019718, 12.50000000000000000, 6.495190528383297135 ) ) ;
#69780=DIRECTION ( 'NONE',  ( 0.000000000000000000, 0.000000000000000000, -1.000000000000000000 ) ) ;
#69781=ADVANCED_FACE ( 'NONE', ( #57264 ), #51489, .T. ) ;
#69782=CARTESIAN_POINT ( 'NONE',  ( -2.100000000000033840, 12.50000000000000000, 3.637306695894644726 ) ) ;
#69783=EDGE_CURVE ( 'NONE', #3939, #69598, #30851, .T. ) ;
#69784=ORIENTED_EDGE ( 'NONE', *, *, #114864, .F. ) ;
#69785=DIRECTION ( 'NONE',  ( -0.000000000000000000, 1.000000000000000000, -0.000000000000000000 ) ) ;
#69786=EDGE_CURVE ( 'NONE', #32002, #63267, #11761, .T. ) ;
#69787=ORIENTED_EDGE ( 'NONE', *, *, #34431, .T. ) ;
#69788=EDGE_CURVE ( 'NONE', #45708, #11852, #53816, .T. ) ;
#69789=ORIENTED_EDGE ( 'NONE', *, *, #5369, .T. ) ;
#69790=CIRCLE ( 'NONE', #17540, 0.1000000000000002554 ) ;
#69791=AXIS2_PLACEMENT_3D ( 'NONE', #6424, #5799, #56196 ) ;
#69792=EDGE_CURVE ( 'NONE', #59157, #29817, #112165, .T. ) ;
#69793=DIRECTION ( 'NONE',  ( -0.000000000000000000, 1.000000000000000000, -0.000000000000000000 ) ) ;
#69794=LINE ( 'NONE', #79614, #92985 ) ;
#69795=CARTESIAN_POINT ( 'NONE',  ( -8.150000000000009237, 2.500000000000000000, 6.941600689897073018 ) ) ;
#69796=ADVANCED_FACE ( 'NONE', ( #119387 ), #81008, .T. ) ;
#69798=DIRECTION ( 'NONE',  ( 0.000000000000000000, 0.000000000000000000, 1.000000000000000000 ) ) ;
#69799=CARTESIAN_POINT ( 'NONE',  ( 4.599999999999936584, 2.500000000000000000, 3.737306695894644371 ) ) ;
#69800=AXIS2_PLACEMENT_3D ( 'NONE', #110874, #49411, #21211 ) ;
#69801=AXIS2_PLACEMENT_3D ( 'NONE', #90730, #394, #121462 ) ;
#69802=CARTESIAN_POINT ( 'NONE',  ( -3.950000000000024603, 2.500000000000000000, 1.718653347947321386 ) ) ;
#69803=CONICAL_SURFACE ( 'NONE', #44768, 0.09999999999999982514, 0.003490658503988666988 ) ;
#69804=DIRECTION ( 'NONE',  ( 0.000000000000000000, 0.000000000000000000, 1.000000000000000000 ) ) ;
#69805=FACE_OUTER_BOUND ( 'NONE', #117728, .T. ) ;
#69806=CIRCLE ( 'NONE', #28037, 0.1000000000000002554 ) ;
#69807=VECTOR ( 'NONE', #17118, 1000.000000000000000 ) ;
#69808=ADVANCED_FACE ( 'NONE', ( #2190 ), #70346, .T. ) ;
#69809=CIRCLE ( 'NONE', #13358, 0.1000000000000002554 ) ;
#69810=VECTOR ( 'NONE', #64783, 1000.000000000000000 ) ;
#69811=VECTOR ( 'NONE', #70196, 1000.000000000000000 ) ;
#69812=ORIENTED_EDGE ( 'NONE', *, *, #58127, .T. ) ;
#69813=DIRECTION ( 'NONE',  ( 0.000000000000000000, 0.000000000000000000, 1.000000000000000000 ) ) ;
#69814=AXIS2_PLACEMENT_3D ( 'NONE', #79926, #11824, #30206 ) ;
#69815=CARTESIAN_POINT ( 'NONE',  ( 6.649999999999929301, 12.50000000000000000, 6.430097255199259010 ) ) ;
#69816=DIRECTION ( 'NONE',  ( 0.000000000000000000, 0.000000000000000000, 1.000000000000000000 ) ) ;
#69818=CARTESIAN_POINT ( 'NONE',  ( -9.200000000000006395, 2.500000000000000000, -2.385244779468109755E-15 ) ) ;
#69819=EDGE_LOOP ( 'NONE', ( #49567, #36229 ) ) ;
#69820=LINE ( 'NONE', #28614, #653 ) ;
#69821=DIRECTION ( 'NONE',  ( 0.000000000000000000, 1.000000000000000000, 0.000000000000000000 ) ) ;
#69822=DIRECTION ( 'NONE',  ( -0.000000000000000000, 1.000000000000000000, -0.000000000000000000 ) ) ;
#69823=EDGE_LOOP ( 'NONE', ( #33543, #79424 ) ) ;
#69824=ADVANCED_FACE ( 'NONE', ( #81423 ), #43180, .T. ) ;
#69825=AXIS2_PLACEMENT_3D ( 'NONE', #87065, #85133, #125067 ) ;
#69826=EDGE_LOOP ( 'NONE', ( #107730, #89909, #95654, #46052 ) ) ;
#69827=CARTESIAN_POINT ( 'NONE',  ( 8.299999999999922551, 2.500000000000000000, 0.09999999999999761857 ) ) ;
#69828=EDGE_LOOP ( 'NONE', ( #4699, #113957, #79270, #90265 ) ) ;
#69829=EDGE_LOOP ( 'NONE', ( #18794, #33884 ) ) ;
#69830=ORIENTED_EDGE ( 'NONE', *, *, #116951, .F. ) ;
#69831=DIRECTION ( 'NONE',  ( -0.000000000000000000, 1.000000000000000000, -0.000000000000000000 ) ) ;
#69833=ADVANCED_FACE ( 'NONE', ( #1399 ), #49439, .T. ) ;
#69834=CARTESIAN_POINT ( 'NONE',  ( -2.900000000000029221, 12.50000000000000000, -2.276824562219559311E-15 ) ) ;
#69835=DIRECTION ( 'NONE',  ( 0.000000000000000000, -0.9999939076577903929, 0.003490651415223739937 ) ) ;
#69836=EDGE_CURVE ( 'NONE', #94563, #62072, #93334, .T. ) ;
#69837=AXIS2_PLACEMENT_3D ( 'NONE', #15106, #84526, #73408 ) ;
#69838=CARTESIAN_POINT ( 'NONE',  ( -3.950000000000024603, 2.500000000000000000, 1.818653347947321475 ) ) ;
#69839=CIRCLE ( 'NONE', #59399, 0.1000000000000000472 ) ;
#69840=ORIENTED_EDGE ( 'NONE', *, *, #100547, .F. ) ;
#69841=EDGE_CURVE ( 'NONE', #18837, #110767, #122587, .T. ) ;
#69843=ORIENTED_EDGE ( 'NONE', *, *, #118613, .T. ) ;
#69844=DIRECTION ( 'NONE',  ( -0.000000000000000000, -1.000000000000000000, -0.000000000000000000 ) ) ;
#69845=PLANE ( 'NONE',  #65252 ) ;
#69846=EDGE_CURVE ( 'NONE', #108066, #126779, #80823, .T. ) ;
#69847=FACE_OUTER_BOUND ( 'NONE', #76881, .T. ) ;
#69848=AXIS2_PLACEMENT_3D ( 'NONE', #64546, #24633, #126037 ) ;
#69849=ADVANCED_FACE ( 'NONE', ( #40713 ), #76610, .T. ) ;
#69850=ORIENTED_EDGE ( 'NONE', *, *, #107198, .T. ) ;
#69851=EDGE_CURVE ( 'NONE', #66462, #73593, #78686, .T. ) ;
#69852=ADVANCED_FACE ( 'NONE', ( #61630 ), #112127, .T. ) ;
#69853=EDGE_LOOP ( 'NONE', ( #47351, #32566 ) ) ;
#69854=EDGE_LOOP ( 'NONE', ( #104495, #15765 ) ) ;
#69855=ORIENTED_EDGE ( 'NONE', *, *, #69836, .F. ) ;
#69856=VERTEX_POINT ( 'NONE', #121817 ) ;
#69857=FACE_OUTER_BOUND ( 'NONE', #46782, .T. ) ;
#69858=FACE_OUTER_BOUND ( 'NONE', #112045, .T. ) ;
#69859=DIRECTION ( 'NONE',  ( -0.000000000000000000, -1.000000000000000000, -0.000000000000000000 ) ) ;
#69860=FACE_BOUND ( 'NONE', #80396, .T. ) ;
#69861=CARTESIAN_POINT ( 'NONE',  ( -5.850000000000021849, 2.500000000000000000, -1.472243186433550122 ) ) ;
#69863=EDGE_CURVE ( 'NONE', #47998, #91773, #13901, .T. ) ;
#69864=CARTESIAN_POINT ( 'NONE',  ( -8.950000000000008171, 12.50000000000000000, -2.511473670974877948 ) ) ;
#69865=DIRECTION ( 'NONE',  ( 0.000000000000000000, 0.000000000000000000, 1.000000000000000000 ) ) ;
#69866=AXIS2_PLACEMENT_3D ( 'NONE', #52336, #81782, #60868 ) ;
#69867=VECTOR ( 'NONE', #40316, 1000.000000000000000 ) ;
#69868=DIRECTION ( 'NONE',  ( 0.000000000000000000, 1.000000000000000000, 0.000000000000000000 ) ) ;
#69869=DIRECTION ( 'NONE',  ( 0.000000000000000000, -0.000000000000000000, 1.000000000000000000 ) ) ;
#69870=CIRCLE ( 'NONE', #15471, 0.1000000000000002554 ) ;
#69871=DIRECTION ( 'NONE',  ( 0.000000000000000000, -0.9999939076577903929, 0.003490651415223739937 ) ) ;
#69872=AXIS2_PLACEMENT_3D ( 'NONE', #67239, #129456, #119589 ) ;
#69873=DIRECTION ( 'NONE',  ( 0.000000000000000000, 0.000000000000000000, -1.000000000000000000 ) ) ;
#69874=EDGE_LOOP ( 'NONE', ( #96932, #50562 ) ) ;
#69875=ORIENTED_EDGE ( 'NONE', *, *, #128329, .T. ) ;
#69876=EDGE_LOOP ( 'NONE', ( #43151, #62592 ) ) ;
#69877=VERTEX_POINT ( 'NONE', #120540 ) ;
#69878=CARTESIAN_POINT ( 'NONE',  ( -11.64999999999999858, 2.500000000000000000, -5.702370205355745902 ) ) ;
#69879=DIRECTION ( 'NONE',  ( 0.000000000000000000, 0.000000000000000000, -1.000000000000000000 ) ) ;
#69880=FACE_BOUND ( 'NONE', #33267, .T. ) ;
#69881=DIRECTION ( 'NONE',  ( -0.000000000000000000, -1.000000000000000000, -0.000000000000000000 ) ) ;
#69882=CONICAL_SURFACE ( 'NONE', #80355, 0.1000000000000002554, 0.003490658503988666988 ) ;
#69883=AXIS2_PLACEMENT_3D ( 'NONE', #112467, #34562, #24078 ) ;
#69884=CIRCLE ( 'NONE', #84554, 0.09999999999999982514 ) ;
#69885=EDGE_LOOP ( 'NONE', ( #972, #9870, #111198, #38559 ) ) ;
#69886=CARTESIAN_POINT ( 'NONE',  ( -4.999999999999986677, 2.500000000000000000, 4.230127018922196669 ) ) ;
#69887=CIRCLE ( 'NONE', #67821, 0.06509327318403745899 ) ;
#69888=DIRECTION ( 'NONE',  ( 0.000000000000000000, 0.000000000000000000, 1.000000000000000000 ) ) ;
#69889=DIRECTION ( 'NONE',  ( -0.000000000000000000, 1.000000000000000000, -0.000000000000000000 ) ) ;
#69890=DIRECTION ( 'NONE',  ( 0.000000000000000000, 1.000000000000000000, 0.000000000000000000 ) ) ;
#69891=ORIENTED_EDGE ( 'NONE', *, *, #24558, .F. ) ;
#69892=DIRECTION ( 'NONE',  ( 0.000000000000000000, 0.000000000000000000, 1.000000000000000000 ) ) ;
#69893=AXIS2_PLACEMENT_3D ( 'NONE', #98319, #116680, #17157 ) ;
#69894=AXIS2_PLACEMENT_3D ( 'NONE', #113734, #81681, #62062 ) ;
#69895=EDGE_CURVE ( 'NONE', #91108, #19600, #20173, .T. ) ;
#69896=VECTOR ( 'NONE', #70309, 1000.000000000000000 ) ;
#69897=ORIENTED_EDGE ( 'NONE', *, *, #19974, .F. ) ;
#69898=ORIENTED_EDGE ( 'NONE', *, *, #51171, .T. ) ;
#69899=DIRECTION ( 'NONE',  ( -0.000000000000000000, -1.000000000000000000, -0.000000000000000000 ) ) ;
#69900=CARTESIAN_POINT ( 'NONE',  ( -6.650000000000014566, 2.500000000000000000, 6.495190528383297135 ) ) ;
#69901=ORIENTED_EDGE ( 'NONE', *, *, #30221, .F. ) ;
#69902=VECTOR ( 'NONE', #101994, 1000.000000000000000 ) ;
#69903=DIRECTION ( 'NONE',  ( -0.000000000000000000, -1.000000000000000000, -0.000000000000000000 ) ) ;
#69904=DIRECTION ( 'NONE',  ( -0.000000000000000000, -1.000000000000000000, -0.000000000000000000 ) ) ;
#69905=ORIENTED_EDGE ( 'NONE', *, *, #54538, .F. ) ;
#69906=CARTESIAN_POINT ( 'NONE',  ( 4.599999999999938360, 2.500000000000000000, 0.09999999999999772959 ) ) ;
#69907=VECTOR ( 'NONE', #10387, 1000.000000000000000 ) ;
#69908=ORIENTED_EDGE ( 'NONE', *, *, #42967, .T. ) ;
#69909=EDGE_CURVE ( 'NONE', #23517, #42124, #31515, .T. ) ;
#69910=PLANE ( 'NONE',  #103873 ) ;
#69911=ORIENTED_EDGE ( 'NONE', *, *, #59367, .F. ) ;
#69912=DIRECTION ( 'NONE',  ( 0.000000000000000000, 0.000000000000000000, 1.000000000000000000 ) ) ;
#69913=ORIENTED_EDGE ( 'NONE', *, *, #52007, .F. ) ;
#69915=ORIENTED_EDGE ( 'NONE', *, *, #95772, .F. ) ;
#69916=DIRECTION ( 'NONE',  ( 0.000000000000000000, 0.000000000000000000, 1.000000000000000000 ) ) ;
#69917=DIRECTION ( 'NONE',  ( 0.000000000000000000, 0.000000000000000000, -1.000000000000000000 ) ) ;
#69918=CARTESIAN_POINT ( 'NONE',  ( 10.19999999999991225, 12.50000000000000000, 3.983716857408420076 ) ) ;
#69919=FACE_OUTER_BOUND ( 'NONE', #32238, .T. ) ;
#69920=CARTESIAN_POINT ( 'NONE',  ( 16.55874544816229488, 0.4845305829427787869, -6.091953208798931207 ) ) ;
#69921=AXIS2_PLACEMENT_3D ( 'NONE', #120192, #90724, #30540 ) ;
#69922=ORIENTED_EDGE ( 'NONE', *, *, #23869, .F. ) ;
#69923=EDGE_LOOP ( 'NONE', ( #52071, #1499, #61163, #82737 ) ) ;
#69924=ORIENTED_EDGE ( 'NONE', *, *, #84207, .F. ) ;
#69925=DIRECTION ( 'NONE',  ( 0.000000000000000000, -0.000000000000000000, 1.000000000000000000 ) ) ;
#69926=DIRECTION ( 'NONE',  ( -4.274815082592931898E-19, -0.9999939076577903929, -0.003490651415223739937 ) ) ;
#69927=CARTESIAN_POINT ( 'NONE',  ( -4.119968255444916849E-14, 12.50000000000000000, 3.637306695894644726 ) ) ;
#69928=EDGE_LOOP ( 'NONE', ( #51277, #62857 ) ) ;
#69929=ORIENTED_EDGE ( 'NONE', *, *, #10791, .T. ) ;
#69930=ORIENTED_EDGE ( 'NONE', *, *, #41317, .T. ) ;
#69931=DIRECTION ( 'NONE',  ( 0.000000000000000000, 0.000000000000000000, 1.000000000000000000 ) ) ;
#69932=AXIS2_PLACEMENT_3D ( 'NONE', #108990, #59936, #321 ) ;
#69933=ORIENTED_EDGE ( 'NONE', *, *, #121357, .T. ) ;
#69934=FACE_OUTER_BOUND ( 'NONE', #99959, .T. ) ;
#69935=AXIS2_PLACEMENT_3D ( 'NONE', #11739, #3851, #64065 ) ;
#69936=EDGE_CURVE ( 'NONE', #49883, #58319, #71416, .T. ) ;
#69938=DIRECTION ( 'NONE',  ( 0.000000000000000000, 1.000000000000000000, 0.000000000000000000 ) ) ;
#69939=CARTESIAN_POINT ( 'NONE',  ( -6.850000000000017408, 2.500000000000000000, -2.611473670974877592 ) ) ;
#69940=CARTESIAN_POINT ( 'NONE',  ( 1.899999999999949507, 2.500000000000000000, 3.883716857408421319 ) ) ;
#69941=DIRECTION ( 'NONE',  ( 0.000000000000000000, 0.000000000000000000, 1.000000000000000000 ) ) ;
#69942=DIRECTION ( 'NONE',  ( 0.000000000000000000, 0.000000000000000000, -1.000000000000000000 ) ) ;
#69943=FACE_OUTER_BOUND ( 'NONE', #60794, .T. ) ;
#69944=EDGE_CURVE ( 'NONE', #78169, #63386, #29575, .T. ) ;
#69945=EDGE_LOOP ( 'NONE', ( #8888, #73613, #41740, #35750 ) ) ;
#69946=EDGE_LOOP ( 'NONE', ( #37615, #81650, #20315, #94322 ) ) ;
#69947=AXIS2_PLACEMENT_3D ( 'NONE', #10111, #61143, #50059 ) ;
#69948=DIRECTION ( 'NONE',  ( 0.000000000000000000, 0.000000000000000000, 1.000000000000000000 ) ) ;
#69949=AXIS2_PLACEMENT_3D ( 'NONE', #25585, #66164, #46518 ) ;
#69950=EDGE_CURVE ( 'NONE', #78151, #39661, #74550, .T. ) ;
#69951=EDGE_LOOP ( 'NONE', ( #57238, #99765 ) ) ;
#69952=EDGE_CURVE ( 'NONE', #59465, #28605, #124720, .T. ) ;
#69953=ORIENTED_EDGE ( 'NONE', *, *, #117200, .T. ) ;
#69954=EDGE_CURVE ( 'NONE', #13985, #76810, #34869, .T. ) ;
#69956=DIRECTION ( 'NONE',  ( 0.000000000000000000, -0.9999939076577903929, 0.003490651415223739937 ) ) ;
#69957=EDGE_CURVE ( 'NONE', #87658, #39511, #98965, .T. ) ;
#69958=ADVANCED_FACE ( 'NONE', ( #19767 ), #99619, .T. ) ;
#69959=DIRECTION ( 'NONE',  ( 0.000000000000000000, 1.000000000000000000, 0.000000000000000000 ) ) ;
#69960=CARTESIAN_POINT ( 'NONE',  ( -0.8500000000000386136, 2.500000000000000000, 7.188010851410848723 ) ) ;
#69961=AXIS2_PLACEMENT_3D ( 'NONE', #109956, #32052, #100133 ) ;
#69962=CARTESIAN_POINT ( 'NONE',  ( -8.550000000000007816, 12.50000000000000000, 6.148780366869520009 ) ) ;
#69963=CIRCLE ( 'NONE', #124244, 0.06509327318403745899 ) ;
#69964=CARTESIAN_POINT ( 'NONE',  ( -13.94999999999998863, 2.500000000000000000, -1.718653347947323828 ) ) ;
#69965=CARTESIAN_POINT ( 'NONE',  ( 3.749999999999938716, 12.50000000000000000, 7.253104124594885960 ) ) ;
#69966=VECTOR ( 'NONE', #11923, 1000.000000000000000 ) ;
#69967=EDGE_CURVE ( 'NONE', #55060, #80681, #110065, .T. ) ;
#69968=CONICAL_SURFACE ( 'NONE', #61652, 0.09999999999999982514, 0.003490658503988666988 ) ;
#69969=DIRECTION ( 'NONE',  ( 0.000000000000000000, -0.000000000000000000, 1.000000000000000000 ) ) ;
#69970=EDGE_CURVE ( 'NONE', #19230, #121105, #103476, .T. ) ;
#69971=ADVANCED_FACE ( 'NONE', ( #42649 ), #95393, .T. ) ;
#69972=ORIENTED_EDGE ( 'NONE', *, *, #123415, .T. ) ;
#69973=ORIENTED_EDGE ( 'NONE', *, *, #120546, .T. ) ;
#69974=ORIENTED_EDGE ( 'NONE', *, *, #33029, .F. ) ;
#69975=ORIENTED_EDGE ( 'NONE', *, *, #70950, .F. ) ;
#69976=CARTESIAN_POINT ( 'NONE',  ( 14.14999999999989733, 2.500000000000000000, 2.957883832488649389 ) ) ;
#69977=CARTESIAN_POINT ( 'NONE',  ( 10.84999999999990905, 12.50000000000000000, -7.188010851410854052 ) ) ;
#69978=ORIENTED_EDGE ( 'NONE', *, *, #79473, .T. ) ;
#69979=CARTESIAN_POINT ( 'NONE',  ( 9.149999999999916866, 2.500000000000000000, -2.857883832488653741 ) ) ;
#69980=CARTESIAN_POINT ( 'NONE',  ( 4.799999999999934097, 12.50000000000000000, 4.741630453620009789 ) ) ;
#69981=AXIS2_PLACEMENT_3D ( 'NONE', #103122, #110987, #93310 ) ;
#69982=DIRECTION ( 'NONE',  ( 0.000000000000000000, -0.9999939076577903929, 0.003490651415223739937 ) ) ;
#69983=DIRECTION ( 'NONE',  ( 0.000000000000000000, 0.000000000000000000, 1.000000000000000000 ) ) ;
#69984=VERTEX_POINT ( 'NONE', #62907 ) ;
#69985=AXIS2_PLACEMENT_3D ( 'NONE', #27130, #67026, #74301 ) ;
#69986=CONICAL_SURFACE ( 'NONE', #124361, 0.09999999999999999167, 0.003490658503988666988 ) ;
#69987=DIRECTION ( 'NONE',  ( 0.000000000000000000, 0.000000000000000000, -1.000000000000000000 ) ) ;
#69988=DIRECTION ( 'NONE',  ( 0.000000000000000000, 0.000000000000000000, 1.000000000000000000 ) ) ;
#69989=VERTEX_POINT ( 'NONE', #5257 ) ;
#69990=CONICAL_SURFACE ( 'NONE', #93070, 0.09999999999999982514, 0.003490658503988666988 ) ;
#69992=ORIENTED_EDGE ( 'NONE', *, *, #57717, .F. ) ;
#69993=ORIENTED_EDGE ( 'NONE', *, *, #39538, .T. ) ;
#69994=EDGE_LOOP ( 'NONE', ( #68473, #61716 ) ) ;
#69995=CARTESIAN_POINT ( 'NONE',  ( 9.799999999999918998, 2.500000000000000000, -0.3464101615137782364 ) ) ;
#69996=CIRCLE ( 'NONE', #55413, 0.09999999999999982514 ) ;
#69997=CARTESIAN_POINT ( 'NONE',  ( 0.3999999999999628852, 2.500000000000000000, -0.6928203230275520319 ) ) ;
#69998=CARTESIAN_POINT ( 'NONE',  ( 3.299999999999944755, 12.50000000000000000, -4.265033745738164406 ) ) ;
#69999=AXIS2_PLACEMENT_3D ( 'NONE', #11009, #90875, #1205 ) ;
#70000=CIRCLE ( 'NONE', #65776, 0.06509327318403745899 ) ;
#70001=LINE ( 'NONE', #38121, #81542 ) ;
#70002=VECTOR ( 'NONE', #87488, 1000.000000000000000 ) ;
#70003=VERTEX_POINT ( 'NONE', #83822 ) ;
#70004=CARTESIAN_POINT ( 'NONE',  ( -1.050000000000037792, 12.50000000000000000, 1.753560074763284016 ) ) ;
#70005=DIRECTION ( 'NONE',  ( -0.000000000000000000, -1.000000000000000000, -0.000000000000000000 ) ) ;
#70006=CARTESIAN_POINT ( 'NONE',  ( -12.89999999999999147, 12.50000000000000000, 3.572213422710607489 ) ) ;
#70007=CARTESIAN_POINT ( 'NONE',  ( 13.09999999999990195, 2.500000000000000000, 3.883716857408420431 ) ) ;
#70008=EDGE_CURVE ( 'NONE', #2830, #41232, #13787, .T. ) ;
#70009=EDGE_CURVE ( 'NONE', #91773, #47998, #30659, .T. ) ;
#70010=VERTEX_POINT ( 'NONE', #64827 ) ;
#70011=DIRECTION ( 'NONE',  ( 0.000000000000000000, -0.9999939076577903929, 0.003490651415223739937 ) ) ;
#70012=ADVANCED_FACE ( 'NONE', ( #3974 ), #18109, .T. ) ;
#70013=ORIENTED_EDGE ( 'NONE', *, *, #48720, .F. ) ;
#70014=ORIENTED_EDGE ( 'NONE', *, *, #121115, .T. ) ;
#70015=FACE_OUTER_BOUND ( 'NONE', #13511, .T. ) ;
#70016=DIRECTION ( 'NONE',  ( 0.000000000000000000, 0.000000000000000000, 1.000000000000000000 ) ) ;
#70017=FACE_BOUND ( 'NONE', #36226, .T. ) ;
#70018=DIRECTION ( 'NONE',  ( 0.000000000000000000, 0.000000000000000000, 1.000000000000000000 ) ) ;
#70019=AXIS2_PLACEMENT_3D ( 'NONE', #97729, #8055, #87257 ) ;
#70020=DIRECTION ( 'NONE',  ( 0.000000000000000000, 0.000000000000000000, 1.000000000000000000 ) ) ;
#70021=EDGE_CURVE ( 'NONE', #92462, #83779, #33462, .T. ) ;
#70022=LINE ( 'NONE', #9803, #31165 ) ;
#70023=DIRECTION ( 'NONE',  ( -4.274815082592931898E-19, -0.9999939076577903929, -0.003490651415223739937 ) ) ;
#70024=CARTESIAN_POINT ( 'NONE',  ( 2.499999999999983569, 12.50000000000000000, -4.330127018922201643 ) ) ;
#70025=DIRECTION ( 'NONE',  ( 0.000000000000000000, 0.000000000000000000, 1.000000000000000000 ) ) ;
#70026=CARTESIAN_POINT ( 'NONE',  ( 6.899999999999928413, 12.50000000000000000, 4.611443907251934426 ) ) ;
#70027=ORIENTED_EDGE ( 'NONE', *, *, #118917, .T. ) ;
#70028=AXIS2_PLACEMENT_3D ( 'NONE', #46716, #56525, #85973 ) ;
#70029=VECTOR ( 'NONE', #69871, 1000.000000000000000 ) ;
#70030=DIRECTION ( 'NONE',  ( 0.000000000000000000, 0.000000000000000000, 1.000000000000000000 ) ) ;
#70031=DIRECTION ( 'NONE',  ( 0.000000000000000000, 0.000000000000000000, -1.000000000000000000 ) ) ;
#70032=EDGE_LOOP ( 'NONE', ( #24697, #34688, #127228, #20107 ) ) ;
#70033=ORIENTED_EDGE ( 'NONE', *, *, #126524, .F. ) ;
#70034=CARTESIAN_POINT ( 'NONE',  ( -4.800000000000028244, 2.500000000000000000, -4.083716857408426826 ) ) ;
#70035=CARTESIAN_POINT ( 'NONE',  ( -0.6000000000000383915, 2.500000000000000000, -4.776537180435977525 ) ) ;
#70036=EDGE_CURVE ( 'NONE', #115297, #95313, #89129, .T. ) ;
#70037=FACE_BOUND ( 'NONE', #45141, .T. ) ;
#70038=LINE ( 'NONE', #69374, #51448 ) ;
#70039=AXIS2_PLACEMENT_3D ( 'NONE', #28308, #37497, #66293 ) ;
#70040=CARTESIAN_POINT ( 'NONE',  ( -11.89999999999999503, 2.500000000000000000, 4.676537180435972552 ) ) ;
#70041=AXIS2_PLACEMENT_3D ( 'NONE', #102083, #90972, #11760 ) ;
#70043=CARTESIAN_POINT ( 'NONE',  ( -10.40000000000000213, 2.500000000000000000, 0.09999999999999772959 ) ) ;
#70044=FACE_OUTER_BOUND ( 'NONE', #52674, .T. ) ;
#70046=DIRECTION ( 'NONE',  ( -0.000000000000000000, -1.000000000000000000, -0.000000000000000000 ) ) ;
#70047=CARTESIAN_POINT ( 'NONE',  ( -9.550000000000006040, 12.50000000000000000, -2.099970236277064473 ) ) ;
#70048=CIRCLE ( 'NONE', #7336, 0.1000000000000000472 ) ;
#70049=ADVANCED_FACE ( 'NONE', ( #43925 ), #116302, .T. ) ;
#70050=CARTESIAN_POINT ( 'NONE',  ( 8.549999999999922551, 2.500000000000000000, -6.248780366869526759 ) ) ;
#70051=PLANE ( 'NONE',  #48857 ) ;
#70052=ORIENTED_EDGE ( 'NONE', *, *, #67744, .T. ) ;
#70053=CARTESIAN_POINT ( 'NONE',  ( 14.19999999999989626, 12.50000000000000000, -2.276824562219559311E-15 ) ) ;
#70054=CARTESIAN_POINT ( 'NONE',  ( 4.599999999999939249, 12.50000000000000000, -3.637306695894650055 ) ) ;
#70055=DIRECTION ( 'NONE',  ( -4.274815082592931898E-19, -0.9999939076577903929, -0.003490651415223739937 ) ) ;
#70056=CARTESIAN_POINT ( 'NONE',  ( 21.24748443165276512, -0.7426079187842464790, -4.181982372968835904 ) ) ;
#70057=VERTEX_POINT ( 'NONE', #112013 ) ;
#70058=ORIENTED_EDGE ( 'NONE', *, *, #9276, .F. ) ;
#70059=EDGE_CURVE ( 'NONE', #111925, #106111, #66134, .T. ) ;
#70060=CARTESIAN_POINT ( 'NONE',  ( 1.649999999999948841, 2.500000000000000000, 6.495190528383297135 ) ) ;
#70061=CIRCLE ( 'NONE', #93051, 0.06509327318403743123 ) ;
#70062=ORIENTED_EDGE ( 'NONE', *, *, #117457, .F. ) ;
#70063=DIRECTION ( 'NONE',  ( 0.000000000000000000, 0.000000000000000000, 1.000000000000000000 ) ) ;
#70065=AXIS2_PLACEMENT_3D ( 'NONE', #988, #70373, #119457 ) ;
#70066=DIRECTION ( 'NONE',  ( 0.000000000000000000, 1.000000000000000000, 0.000000000000000000 ) ) ;
#70067=ORIENTED_EDGE ( 'NONE', *, *, #120671, .T. ) ;
#70068=CONICAL_SURFACE ( 'NONE', #34582, 0.1000000000000000472, 0.003490658503988666988 ) ;
#70069=CARTESIAN_POINT ( 'NONE',  ( -8.100000000000013856, 2.500000000000000000, -0.4464101615137782142 ) ) ;
#70070=FACE_OUTER_BOUND ( 'NONE', #61286, .T. ) ;
#70071=CARTESIAN_POINT ( 'NONE',  ( 87.50000000000001421, 3.974992050023850698, -6.359987280038159163 ) ) ;
#70072=VECTOR ( 'NONE', #95034, 1000.000000000000000 ) ;
#70073=DIRECTION ( 'NONE',  ( 0.000000000000000000, 0.000000000000000000, -1.000000000000000000 ) ) ;
#70074=PLANE ( 'NONE',  #82104 ) ;
#70075=DIRECTION ( 'NONE',  ( 0.000000000000000000, 1.000000000000000000, 0.000000000000000000 ) ) ;
#70076=CIRCLE ( 'NONE', #38711, 0.06509327318403743123 ) ;
#70077=EDGE_LOOP ( 'NONE', ( #108893, #96201, #124793, #111638 ) ) ;
#70078=AXIS2_PLACEMENT_3D ( 'NONE', #22763, #71188, #72498 ) ;
#70079=ORIENTED_EDGE ( 'NONE', *, *, #29320, .T. ) ;
#70080=AXIS2_PLACEMENT_3D ( 'NONE', #98272, #47907, #126464 ) ;
#70081=CARTESIAN_POINT ( 'NONE',  ( 4.599999999999935696, 12.50000000000000000, 5.022947341949748790 ) ) ;
#70082=EDGE_LOOP ( 'NONE', ( #18040, #110042 ) ) ;
#70083=CARTESIAN_POINT ( 'NONE',  ( -7.700000000000012612, 2.500000000000000000, 4.576537180435972019 ) ) ;
#70084=CONICAL_SURFACE ( 'NONE', #118195, 0.09999999999999982514, 0.003490658503988666988 ) ;
#70085=ORIENTED_EDGE ( 'NONE', *, *, #16994, .F. ) ;
#70086=ORIENTED_EDGE ( 'NONE', *, *, #24124, .T. ) ;
#70087=ORIENTED_EDGE ( 'NONE', *, *, #63918, .T. ) ;
#70088=CARTESIAN_POINT ( 'NONE',  ( 87.50000000000000000, -0.7169905660282998028, -7.499999999999998224 ) ) ;
#70089=AXIS2_PLACEMENT_3D ( 'NONE', #73018, #102477, #12786 ) ;
#70090=DIRECTION ( 'NONE',  ( 0.000000000000000000, 0.000000000000000000, -1.000000000000000000 ) ) ;
#70091=AXIS2_PLACEMENT_3D ( 'NONE', #53323, #53956, #13376 ) ;
#70092=CARTESIAN_POINT ( 'NONE',  ( 11.64999999999990443, 2.500000000000000000, -7.188010851410854052 ) ) ;
#70093=EDGE_CURVE ( 'NONE', #17252, #96946, #99605, .T. ) ;
#70095=DIRECTION ( 'NONE',  ( 0.000000000000000000, 0.000000000000000000, -1.000000000000000000 ) ) ;
#70096=LINE ( 'NONE', #51110, #121233 ) ;
#70097=DIRECTION ( 'NONE',  ( 0.000000000000000000, 0.000000000000000000, 1.000000000000000000 ) ) ;
#70098=CARTESIAN_POINT ( 'NONE',  ( -7.900000000000014566, 12.50000000000000000, 0.06509327318403515528 ) ) ;
#70099=CARTESIAN_POINT ( 'NONE',  ( 0.8499999999999527933, 2.500000000000000000, 7.188010851410848723 ) ) ;
#70100=LINE ( 'NONE', #79913, #35220 ) ;
#70101=ORIENTED_EDGE ( 'NONE', *, *, #104618, .F. ) ;
#70102=ADVANCED_FACE ( 'NONE', ( #85112 ), #9711, .T. ) ;
#70103=EDGE_LOOP ( 'NONE', ( #48747, #62470 ) ) ;
#70104=CARTESIAN_POINT ( 'NONE',  ( 10.64999999999991331, 2.500000000000000000, -1.818653347947325916 ) ) ;
#70105=EDGE_CURVE ( 'NONE', #33814, #1760, #125039, .T. ) ;
#70106=ORIENTED_EDGE ( 'NONE', *, *, #31896, .T. ) ;
#70107=EDGE_CURVE ( 'NONE', #11509, #103770, #82973, .T. ) ;
#70108=ORIENTED_EDGE ( 'NONE', *, *, #73831, .F. ) ;
#70109=EDGE_CURVE ( 'NONE', #102432, #66032, #62274, .T. ) ;
#70110=CARTESIAN_POINT ( 'NONE',  ( 0.6499999999999543920, 2.500000000000000000, 6.148780366869520897 ) ) ;
#70111=EDGE_CURVE ( 'NONE', #83056, #17094, #24470, .T. ) ;
#70112=CIRCLE ( 'NONE', #82733, 0.06509327318403745899 ) ;
#70113=FACE_OUTER_BOUND ( 'NONE', #92076, .T. ) ;
#70114=CARTESIAN_POINT ( 'NONE',  ( -4.350000000000023626, 2.500000000000000000, 6.048780366869521252 ) ) ;
#70115=DIRECTION ( 'NONE',  ( -4.274815082592931898E-19, -0.9999939076577903929, -0.003490651415223739937 ) ) ;
#70116=CARTESIAN_POINT ( 'NONE',  ( -1.700000000000034817, 12.50000000000000000, -4.265033745738164406 ) ) ;
#70117=EDGE_CURVE ( 'NONE', #43052, #28988, #32821, .T. ) ;
#70118=LINE ( 'NONE', #110041, #109532 ) ;
#70119=ORIENTED_EDGE ( 'NONE', *, *, #22714, .F. ) ;
#70120=EDGE_CURVE ( 'NONE', #63981, #31023, #114346, .T. ) ;
#70121=CIRCLE ( 'NONE', #13658, 0.09999999999999999167 ) ;
#70122=ADVANCED_FACE ( 'NONE', ( #127622 ), #60005, .T. ) ;
#70123=AXIS2_PLACEMENT_3D ( 'NONE', #33802, #54091, #37035 ) ;
#70124=EDGE_CURVE ( 'NONE', #37517, #31757, #47456, .T. ) ;
#70125=VERTEX_POINT ( 'NONE', #115192 ) ;
#70126=FACE_OUTER_BOUND ( 'NONE', #7133, .T. ) ;
#70127=EDGE_CURVE ( 'NONE', #41488, #103678, #89222, .T. ) ;
#70128=ORIENTED_EDGE ( 'NONE', *, *, #129559, .F. ) ;
#70129=DIRECTION ( 'NONE',  ( 0.000000000000000000, 1.000000000000000000, 0.000000000000000000 ) ) ;
#70130=EDGE_LOOP ( 'NONE', ( #20812, #44427, #26668, #61074 ) ) ;
#70131=ORIENTED_EDGE ( 'NONE', *, *, #29806, .T. ) ;
#70132=EDGE_CURVE ( 'NONE', #54614, #52844, #53710, .T. ) ;
#70133=DIRECTION ( 'NONE',  ( 0.000000000000000000, 0.000000000000000000, -1.000000000000000000 ) ) ;
#70134=CARTESIAN_POINT ( 'NONE',  ( 4.999999999999971578, 2.500000000000000000, 0.09999999999999772959 ) ) ;
#70135=AXIS2_PLACEMENT_3D ( 'NONE', #68864, #79352, #108783 ) ;
#70136=DIRECTION ( 'NONE',  ( 0.000000000000000000, 0.000000000000000000, -1.000000000000000000 ) ) ;
#70137=DIRECTION ( 'NONE',  ( -4.274815082592931898E-19, -0.9999939076577903929, -0.003490651415223739937 ) ) ;
#70138=CONICAL_SURFACE ( 'NONE', #86844, 0.1000000000000002554, 0.003490658503988666988 ) ;
#70139=FACE_OUTER_BOUND ( 'NONE', #109739, .T. ) ;
#70140=EDGE_LOOP ( 'NONE', ( #101041, #77012, #124739, #55821 ) ) ;
#70141=LINE ( 'NONE', #20390, #37384 ) ;
#70142=DIRECTION ( 'NONE',  ( 0.000000000000000000, 1.000000000000000000, 0.000000000000000000 ) ) ;
#70143=DIRECTION ( 'NONE',  ( -0.000000000000000000, -1.000000000000000000, -0.000000000000000000 ) ) ;
#70144=DIRECTION ( 'NONE',  ( 0.000000000000000000, 1.000000000000000000, 0.000000000000000000 ) ) ;
#70145=DIRECTION ( 'NONE',  ( 0.000000000000000000, 0.000000000000000000, 1.000000000000000000 ) ) ;
#70146=VERTEX_POINT ( 'NONE', #27467 ) ;
#70147=VECTOR ( 'NONE', #87240, 1000.000000000000000 ) ;
#70148=CIRCLE ( 'NONE', #63875, 0.09999999999999982514 ) ;
#70149=VERTEX_POINT ( 'NONE', #86396 ) ;
#70150=CARTESIAN_POINT ( 'NONE',  ( 3.149999999999946176, 12.50000000000000000, -6.148780366869526226 ) ) ;
#70151=EDGE_CURVE ( 'NONE', #23957, #64139, #68053, .T. ) ;
#70152=ORIENTED_EDGE ( 'NONE', *, *, #21341, .T. ) ;
#70153=CARTESIAN_POINT ( 'NONE',  ( 17.50011966276722930, -2.224296756944748488, 4.070989939658955947 ) ) ;
#70154=CARTESIAN_POINT ( 'NONE',  ( -11.64999999999999680, 2.500000000000000000, 7.288010851410849256 ) ) ;
#70155=VECTOR ( 'NONE', #63310, 1000.000000000000000 ) ;
#70156=ORIENTED_EDGE ( 'NONE', *, *, #59767, .T. ) ;
#70157=DIRECTION ( 'NONE',  ( -0.000000000000000000, 1.000000000000000000, -0.000000000000000000 ) ) ;
#70158=CARTESIAN_POINT ( 'NONE',  ( -2.100000000000034728, 2.500000000000000000, 4.230127018922196669 ) ) ;
#70159=CARTESIAN_POINT ( 'NONE',  ( -3.749999999999994671, 2.500000000000000000, -6.595190528383302109 ) ) ;
#70160=AXIS2_PLACEMENT_3D ( 'NONE', #127569, #6463, #46418 ) ;
#70161=DIRECTION ( 'NONE',  ( 0.000000000000000000, -0.9999939076577903929, 0.003490651415223739937 ) ) ;
#70162=EDGE_CURVE ( 'NONE', #73210, #109722, #16036, .T. ) ;
#70163=AXIS2_PLACEMENT_3D ( 'NONE', #62507, #33050, #72321 ) ;
#70164=DIRECTION ( 'NONE',  ( 0.000000000000000000, 1.000000000000000000, 0.000000000000000000 ) ) ;
#70165=CIRCLE ( 'NONE', #103617, 0.06509327318403745899 ) ;
#70166=ADVANCED_FACE ( 'NONE', ( #18305 ), #122666, .T. ) ;
#70167=ORIENTED_EDGE ( 'NONE', *, *, #78989, .F. ) ;
#70168=CARTESIAN_POINT ( 'NONE',  ( -4.350000000000023626, 12.50000000000000000, 2.511473670974873507 ) ) ;
#70169=CARTESIAN_POINT ( 'NONE',  ( -8.550000000000014921, 2.500000000000000000, -6.048780366869521252 ) ) ;
#70170=EDGE_CURVE ( 'NONE', #99317, #95559, #22339, .T. ) ;
#70171=VERTEX_POINT ( 'NONE', #26845 ) ;
#70172=CONICAL_SURFACE ( 'NONE', #34685, 0.1000000000000000472, 0.003490658503988666988 ) ;
#70173=EDGE_LOOP ( 'NONE', ( #34865, #63035 ) ) ;
#70174=CARTESIAN_POINT ( 'NONE',  ( 8.149999999999920419, 2.500000000000000000, 6.741600689897071952 ) ) ;
#70175=DIRECTION ( 'NONE',  ( 0.000000000000000000, -0.9999939076577903929, 0.003490651415223739937 ) ) ;
#70176=CARTESIAN_POINT ( 'NONE',  ( 0.3999999999999628852, 2.500000000000000000, 0.6928203230275518099 ) ) ;
#70177=VERTEX_POINT ( 'NONE', #98152 ) ;
#70178=AXIS2_PLACEMENT_3D ( 'NONE', #108274, #98438, #8763 ) ;
#70179=VECTOR ( 'NONE', #8692, 1000.000000000000000 ) ;
#70180=DIRECTION ( 'NONE',  ( 0.000000000000000000, 0.000000000000000000, 1.000000000000000000 ) ) ;
#70181=AXIS2_PLACEMENT_3D ( 'NONE', #39525, #109530, #121277 ) ;
#70182=CARTESIAN_POINT ( 'NONE',  ( 3.749999999999976907, 2.500000000000000000, 2.265063509461097357 ) ) ;
#70183=VECTOR ( 'NONE', #68681, 1000.000000000000000 ) ;
#70185=DIRECTION ( 'NONE',  ( -0.000000000000000000, 1.000000000000000000, -0.000000000000000000 ) ) ;
#70186=ORIENTED_EDGE ( 'NONE', *, *, #36990, .F. ) ;
#70187=CARTESIAN_POINT ( 'NONE',  ( -3.350000000000031619, 2.500000000000000000, -5.702370205355749455 ) ) ;
#70188=ORIENTED_EDGE ( 'NONE', *, *, #70132, .T. ) ;
#70189=CARTESIAN_POINT ( 'NONE',  ( -11.84999999999999609, 2.500000000000000000, 2.511473670974873507 ) ) ;
#70190=CARTESIAN_POINT ( 'NONE',  ( -4.600000000000028066, 12.50000000000000000, -4.957854068765716882 ) ) ;
#70191=ORIENTED_EDGE ( 'NONE', *, *, #17034, .T. ) ;
#70193=FACE_OUTER_BOUND ( 'NONE', #26054, .T. ) ;
#70194=DIRECTION ( 'NONE',  ( 0.000000000000000000, 0.000000000000000000, 1.000000000000000000 ) ) ;
#70195=ORIENTED_EDGE ( 'NONE', *, *, #63108, .F. ) ;
#70196=DIRECTION ( 'NONE',  ( 0.000000000000000000, -0.9999939076577903929, 0.003490651415223739937 ) ) ;
#70197=EDGE_CURVE ( 'NONE', #7097, #5713, #97628, .T. ) ;
#70198=DIRECTION ( 'NONE',  ( 0.000000000000000000, 0.000000000000000000, 1.000000000000000000 ) ) ;
#70199=CARTESIAN_POINT ( 'NONE',  ( -11.64999999999999680, 12.50000000000000000, 6.495190528383297135 ) ) ;
#70200=DIRECTION ( 'NONE',  ( -0.000000000000000000, -1.000000000000000000, -0.000000000000000000 ) ) ;
#70201=DIRECTION ( 'NONE',  ( 0.000000000000000000, 0.000000000000000000, 1.000000000000000000 ) ) ;
#70202=FACE_OUTER_BOUND ( 'NONE', #45321, .T. ) ;
#70203=CONICAL_SURFACE ( 'NONE', #122444, 0.1000000000000000472, 0.003490658503988666988 ) ;
#70204=CARTESIAN_POINT ( 'NONE',  ( -12.89999999999999147, 2.500000000000000000, 1.843143693225357538E-15 ) ) ;
#70205=CONICAL_SURFACE ( 'NONE', #99463, 0.1000000000000002554, 0.003490658503988666988 ) ;
#70206=CIRCLE ( 'NONE', #128820, 0.06509327318403745899 ) ;
#70207=ORIENTED_EDGE ( 'NONE', *, *, #24608, .F. ) ;
#70208=CIRCLE ( 'NONE', #105807, 0.09999999999999999167 ) ;
#70209=EDGE_LOOP ( 'NONE', ( #97291, #84577 ) ) ;
#70210=VERTEX_POINT ( 'NONE', #88319 ) ;
#70211=DIRECTION ( 'NONE',  ( -4.274815082592931898E-19, -0.9999939076577903929, -0.003490651415223739937 ) ) ;
#70212=CARTESIAN_POINT ( 'NONE',  ( -7.500000000000001776, -1.500000000000000000, 1.734723475976807094E-15 ) ) ;
#70213=ADVANCED_FACE ( 'NONE', ( #106049 ), #57927, .T. ) ;
#70214=DIRECTION ( 'NONE',  ( 0.000000000000000000, 1.000000000000000000, 0.000000000000000000 ) ) ;
#70215=ORIENTED_EDGE ( 'NONE', *, *, #127123, .F. ) ;
#70216=ORIENTED_EDGE ( 'NONE', *, *, #20782, .T. ) ;
#70217=FACE_BOUND ( 'NONE', #59806, .T. ) ;
#70218=VERTEX_POINT ( 'NONE', #36683 ) ;
#70219=ADVANCED_FACE ( 'NONE', ( #97512 ), #108082, .T. ) ;
#70220=FACE_OUTER_BOUND ( 'NONE', #105438, .T. ) ;
#70221=DIRECTION ( 'NONE',  ( 1.000000000000000000, -0.000000000000000000, -0.000000000000000000 ) ) ;
#70222=CARTESIAN_POINT ( 'NONE',  ( 1.449999999999952660, 12.50000000000000000, -6.776507416713040577 ) ) ;
#70223=CARTESIAN_POINT ( 'NONE',  ( 17.99892160975016253, -2.500000000000000000, 4.934975027008865034 ) ) ;
#70224=PLANE ( 'NONE',  #59704 ) ;
#70225=CIRCLE ( 'NONE', #15830, 0.06509327318403743123 ) ;
#70226=AXIS2_PLACEMENT_3D ( 'NONE', #92431, #2759, #101623 ) ;
#70227=DIRECTION ( 'NONE',  ( -0.000000000000000000, 1.000000000000000000, -0.000000000000000000 ) ) ;
#70229=DIRECTION ( 'NONE',  ( 0.000000000000000000, -0.000000000000000000, 1.000000000000000000 ) ) ;
#70230=ADVANCED_FACE ( 'NONE', ( #7837 ), #74638, .T. ) ;
#70231=CARTESIAN_POINT ( 'NONE',  ( 3.549999999999943867, 2.500000000000000000, -6.148780366869526226 ) ) ;
#70232=DIRECTION ( 'NONE',  ( 0.000000000000000000, 0.000000000000000000, -1.000000000000000000 ) ) ;
#70233=AXIS2_PLACEMENT_3D ( 'NONE', #123782, #115911, #56978 ) ;
#70234=ORIENTED_EDGE ( 'NONE', *, *, #22088, .F. ) ;
#70235=ORIENTED_EDGE ( 'NONE', *, *, #100968, .F. ) ;
#70236=VECTOR ( 'NONE', #72165, 1000.000000000000000 ) ;
#70237=ORIENTED_EDGE ( 'NONE', *, *, #101903, .T. ) ;
#70238=ORIENTED_EDGE ( 'NONE', *, *, #59740, .T. ) ;
#70239=CARTESIAN_POINT ( 'NONE',  ( 7.899999999999924860, 2.500000000000000000, 4.230127018922196669 ) ) ;
#70240=CARTESIAN_POINT ( 'NONE',  ( -13.14999999999999147, 2.500000000000000000, 1.918653347947325338 ) ) ;
#70241=ORIENTED_EDGE ( 'NONE', *, *, #30393, .F. ) ;
#70242=ORIENTED_EDGE ( 'NONE', *, *, #42178, .F. ) ;
#70243=ORIENTED_EDGE ( 'NONE', *, *, #75036, .F. ) ;
#70244=LINE ( 'NONE', #59808, #75208 ) ;
#70245=PLANE ( 'NONE',  #105217 ) ;
#70246=FACE_OUTER_BOUND ( 'NONE', #81946, .T. ) ;
#70247=DIRECTION ( 'NONE',  ( -0.000000000000000000, -1.000000000000000000, -0.000000000000000000 ) ) ;
#70248=FACE_OUTER_BOUND ( 'NONE', #3710, .T. ) ;
#70249=LINE ( 'NONE', #110177, #49743 ) ;
#70250=FACE_OUTER_BOUND ( 'NONE', #94259, .T. ) ;
#70251=ORIENTED_EDGE ( 'NONE', *, *, #110213, .T. ) ;
#70252=FACE_OUTER_BOUND ( 'NONE', #118038, .T. ) ;
#70253=VERTEX_POINT ( 'NONE', #56922 ) ;
#70254=EDGE_CURVE ( 'NONE', #1609, #49878, #70446, .T. ) ;
#70255=VECTOR ( 'NONE', #127070, 1000.000000000000000 ) ;
#70256=ORIENTED_EDGE ( 'NONE', *, *, #44210, .T. ) ;
#70257=EDGE_LOOP ( 'NONE', ( #20202, #24180, #127382, #124400 ) ) ;
#70258=AXIS2_PLACEMENT_3D ( 'NONE', #71403, #70144, #2657 ) ;
#70259=CARTESIAN_POINT ( 'NONE',  ( -1.900000000000035438, 2.500000000000000000, 4.083716857408420609 ) ) ;
#70260=EDGE_LOOP ( 'NONE', ( #22600, #29492 ) ) ;
#70261=ADVANCED_FACE ( 'NONE', ( #26204 ), #91369, .T. ) ;
#70262=EDGE_LOOP ( 'NONE', ( #87747, #128106 ) ) ;
#70263=ADVANCED_FACE ( 'NONE', ( #46472 ), #32807, .T. ) ;
#70264=DIRECTION ( 'NONE',  ( -0.000000000000000000, 1.000000000000000000, -0.000000000000000000 ) ) ;
#70265=VECTOR ( 'NONE', #60069, 1000.000000000000000 ) ;
#70267=DIRECTION ( 'NONE',  ( -0.000000000000000000, 1.000000000000000000, -0.000000000000000000 ) ) ;
#70268=DIRECTION ( 'NONE',  ( -0.000000000000000000, -1.000000000000000000, -0.000000000000000000 ) ) ;
#70269=CARTESIAN_POINT ( 'NONE',  ( 4.149999999999938183, 2.500000000000000000, 7.288010851410849256 ) ) ;
#70270=ADVANCED_FACE ( 'NONE', ( #37327 ), #77233, .T. ) ;
#70271=CARTESIAN_POINT ( 'NONE',  ( -2.900000000000030109, 2.500000000000000000, -3.637306695894650055 ) ) ;
#70272=ADVANCED_FACE ( 'NONE', ( #90257 ), #105944, .T. ) ;
#70273=EDGE_CURVE ( 'NONE', #3662, #48633, #85099, .T. ) ;
#70274=ORIENTED_EDGE ( 'NONE', *, *, #23379, .T. ) ;
#70275=DIRECTION ( 'NONE',  ( -0.000000000000000000, -1.000000000000000000, -0.000000000000000000 ) ) ;
#70276=CIRCLE ( 'NONE', #80745, 0.06509327318403745899 ) ;
#70277=VERTEX_POINT ( 'NONE', #19607 ) ;
#70278=CARTESIAN_POINT ( 'NONE',  ( 4.599999999999935696, 12.50000000000000000, 5.088040615133786027 ) ) ;
#70279=AXIS2_PLACEMENT_3D ( 'NONE', #106774, #36123, #105509 ) ;
#70280=EDGE_CURVE ( 'NONE', #75731, #27272, #30756, .T. ) ;
#70281=ORIENTED_EDGE ( 'NONE', *, *, #113997, .T. ) ;
#70282=CARTESIAN_POINT ( 'NONE',  ( -13.09999999999999254, 2.500000000000000000, -0.3464101615137741286 ) ) ;
#70283=DIRECTION ( 'NONE',  ( -0.000000000000000000, -1.000000000000000000, -0.000000000000000000 ) ) ;
#70284=VERTEX_POINT ( 'NONE', #30093 ) ;
#70285=CARTESIAN_POINT ( 'NONE',  ( -11.44999999999999751, 2.500000000000000000, -6.941600689897074794 ) ) ;
#70286=CARTESIAN_POINT ( 'NONE',  ( -11.64999999999999680, 12.50000000000000000, 2.165063509461097713 ) ) ;
#70287=ORIENTED_EDGE ( 'NONE', *, *, #85978, .F. ) ;
#70288=EDGE_CURVE ( 'NONE', #97686, #127904, #59566, .T. ) ;
#70289=FACE_OUTER_BOUND ( 'NONE', #112009, .T. ) ;
#70290=VERTEX_POINT ( 'NONE', #70004 ) ;
#70291=EDGE_LOOP ( 'NONE', ( #2496, #68151, #51413, #87888 ) ) ;
#70292=DIRECTION ( 'NONE',  ( 0.000000000000000000, -0.000000000000000000, 1.000000000000000000 ) ) ;
#70293=DIRECTION ( 'NONE',  ( 0.000000000000000000, 0.000000000000000000, 1.000000000000000000 ) ) ;
#70295=AXIS2_PLACEMENT_3D ( 'NONE', #127534, #37855, #19504 ) ;
#70296=DIRECTION ( 'NONE',  ( 0.000000000000000000, 0.000000000000000000, 1.000000000000000000 ) ) ;
#70297=CARTESIAN_POINT ( 'NONE',  ( -3.749999999999991562, 12.50000000000000000, 6.495190528383297135 ) ) ;
#70299=CONICAL_SURFACE ( 'NONE', #124678, 0.1000000000000000472, 0.003490658503988666988 ) ;
#70300=DIRECTION ( 'NONE',  ( -4.274815082592931898E-19, -0.9999939076577903929, -0.003490651415223739937 ) ) ;
#70301=AXIS2_PLACEMENT_3D ( 'NONE', #85671, #124314, #5167 ) ;
#70302=CIRCLE ( 'NONE', #87015, 0.09999999999999982514 ) ;
#70303=VERTEX_POINT ( 'NONE', #595 ) ;
#70304=CIRCLE ( 'NONE', #114216, 0.1000000000000000056 ) ;
#70305=CARTESIAN_POINT ( 'NONE',  ( 3.549999999999944755, 2.500000000000000000, -6.741600689897077281 ) ) ;
#70306=DIRECTION ( 'NONE',  ( -0.000000000000000000, -1.000000000000000000, -0.000000000000000000 ) ) ;
#70307=AXIS2_PLACEMENT_3D ( 'NONE', #75817, #95470, #17537 ) ;
#70308=DIRECTION ( 'NONE',  ( 0.000000000000000000, 0.000000000000000000, 1.000000000000000000 ) ) ;
#70309=DIRECTION ( 'NONE',  ( -4.274815082592931898E-19, -0.9999939076577903929, -0.003490651415223739937 ) ) ;
#70310=CARTESIAN_POINT ( 'NONE',  ( 12.09999999999990550, 12.50000000000000000, -4.265033745738164406 ) ) ;
#70312=DIRECTION ( 'NONE',  ( 0.000000000000000000, 1.000000000000000000, 0.000000000000000000 ) ) ;
#70313=ORIENTED_EDGE ( 'NONE', *, *, #106421, .F. ) ;
#70314=CIRCLE ( 'NONE', #24247, 0.06509327318403745899 ) ;
#70315=CARTESIAN_POINT ( 'NONE',  ( -8.350000000000012079, 2.500000000000000000, -2.757883832488654097 ) ) ;
#70316=EDGE_CURVE ( 'NONE', #71034, #95476, #31373, .T. ) ;
#70317=VECTOR ( 'NONE', #42406, 1000.000000000000000 ) ;
#70318=AXIS2_PLACEMENT_3D ( 'NONE', #83748, #111246, #34007 ) ;
#70319=DIRECTION ( 'NONE',  ( -0.000000000000000000, -1.000000000000000000, -0.000000000000000000 ) ) ;
#70320=CARTESIAN_POINT ( 'NONE',  ( 9.349999999999919709, 2.500000000000000000, -6.148780366869526226 ) ) ;
#70321=ORIENTED_EDGE ( 'NONE', *, *, #22262, .T. ) ;
#70322=CARTESIAN_POINT ( 'NONE',  ( -6.050000000000017586, 12.50000000000000000, 1.818653347947321475 ) ) ;
#70323=EDGE_CURVE ( 'NONE', #80502, #7747, #112210, .T. ) ;
#70324=VERTEX_POINT ( 'NONE', #11054 ) ;
#70325=ORIENTED_EDGE ( 'NONE', *, *, #47899, .F. ) ;
#70326=CARTESIAN_POINT ( 'NONE',  ( -8.750000000000012434, 2.500000000000000000, -5.902370205355745192 ) ) ;
#70327=ORIENTED_EDGE ( 'NONE', *, *, #49921, .T. ) ;
#70328=DIRECTION ( 'NONE',  ( 0.000000000000000000, 0.000000000000000000, -1.000000000000000000 ) ) ;
#70329=DIRECTION ( 'NONE',  ( -0.000000000000000000, -1.000000000000000000, -0.000000000000000000 ) ) ;
#70330=VERTEX_POINT ( 'NONE', #50354 ) ;
#70331=CARTESIAN_POINT ( 'NONE',  ( 3.299999999999942979, 2.500000000000000000, 4.230127018922196669 ) ) ;
#70332=DIRECTION ( 'NONE',  ( -0.000000000000000000, -1.000000000000000000, -0.000000000000000000 ) ) ;
#70333=CARTESIAN_POINT ( 'NONE',  ( -15.39999999999997904, 2.500000000000000000, -0.7928203230275518987 ) ) ;
#70334=EDGE_LOOP ( 'NONE', ( #65794, #34346 ) ) ;
#70335=CIRCLE ( 'NONE', #47451, 0.06509327318403745899 ) ;
#70336=ORIENTED_EDGE ( 'NONE', *, *, #104756, .T. ) ;
#70337=ORIENTED_EDGE ( 'NONE', *, *, #97544, .F. ) ;
#70338=CARTESIAN_POINT ( 'NONE',  ( 1.249999999999952038, 2.500000000000000000, 2.757883832488649656 ) ) ;
#70339=CARTESIAN_POINT ( 'NONE',  ( 6.899999999999926636, 12.50000000000000000, -0.3464101615137782364 ) ) ;
#70340=DIRECTION ( 'NONE',  ( 0.000000000000000000, 1.000000000000000000, 0.000000000000000000 ) ) ;
#70341=FACE_BOUND ( 'NONE', #13370, .T. ) ;
#70342=EDGE_LOOP ( 'NONE', ( #52345, #21381, #865, #30661 ) ) ;
#70343=DIRECTION ( 'NONE',  ( 0.000000000000000000, 0.000000000000000000, 1.000000000000000000 ) ) ;
#70344=DIRECTION ( 'NONE',  ( -0.000000000000000000, -1.000000000000000000, -0.000000000000000000 ) ) ;
#70345=EDGE_LOOP ( 'NONE', ( #69670, #53746, #112342, #55307 ) ) ;
#70346=CONICAL_SURFACE ( 'NONE', #15947, 0.1000000000000002554, 0.003490658503988666988 ) ;
#70347=AXIS2_PLACEMENT_3D ( 'NONE', #38836, #99012, #79382 ) ;
#70348=DIRECTION ( 'NONE',  ( -0.000000000000000000, -1.000000000000000000, -0.000000000000000000 ) ) ;
#70349=EDGE_CURVE ( 'NONE', #2854, #76377, #55769, .T. ) ;
#70350=LINE ( 'NONE', #89976, #118156 ) ;
#70351=DIRECTION ( 'NONE',  ( -0.000000000000000000, 1.000000000000000000, -0.000000000000000000 ) ) ;
#70352=DIRECTION ( 'NONE',  ( 0.000000000000000000, 0.000000000000000000, 1.000000000000000000 ) ) ;
#70354=CARTESIAN_POINT ( 'NONE',  ( -13.74999999999998757, 12.50000000000000000, -2.857883832488651521 ) ) ;
#70355=DIRECTION ( 'NONE',  ( -0.000000000000000000, 1.000000000000000000, -0.000000000000000000 ) ) ;
#70356=CIRCLE ( 'NONE', #36923, 0.1000000000000002554 ) ;
#70357=CONICAL_SURFACE ( 'NONE', #36924, 0.09999999999999982514, 0.003490658503988666988 ) ;
#70358=EDGE_CURVE ( 'NONE', #75765, #79726, #121028, .T. ) ;
#70359=ORIENTED_EDGE ( 'NONE', *, *, #123589, .F. ) ;
#70360=EDGE_LOOP ( 'NONE', ( #97757, #11141 ) ) ;
#70361=VERTEX_POINT ( 'NONE', #79186 ) ;
#70363=DIRECTION ( 'NONE',  ( -0.000000000000000000, -1.000000000000000000, -0.000000000000000000 ) ) ;
#70364=EDGE_CURVE ( 'NONE', #28471, #118431, #111189, .T. ) ;
#70365=DIRECTION ( 'NONE',  ( 0.000000000000000000, 0.000000000000000000, 1.000000000000000000 ) ) ;
#70366=VERTEX_POINT ( 'NONE', #30740 ) ;
#70367=FACE_BOUND ( 'NONE', #115929, .T. ) ;
#70368=EDGE_CURVE ( 'NONE', #18789, #70557, #21540, .T. ) ;
#70369=DIRECTION ( 'NONE',  ( 0.000000000000000000, 0.000000000000000000, 1.000000000000000000 ) ) ;
#70370=CARTESIAN_POINT ( 'NONE',  ( -8.749999999999975131, 2.500000000000000000, 2.265063509461097357 ) ) ;
#70371=ADVANCED_FACE ( 'NONE', ( #51019 ), #36995, .T. ) ;
#70372=CARTESIAN_POINT ( 'NONE',  ( 6.849999999999930367, 2.500000000000000000, -6.148780366869526226 ) ) ;
#70373=DIRECTION ( 'NONE',  ( -0.000000000000000000, 1.000000000000000000, -0.000000000000000000 ) ) ;
#70374=LINE ( 'NONE', #110298, #32945 ) ;
#70375=DIRECTION ( 'NONE',  ( 0.000000000000000000, 0.000000000000000000, 1.000000000000000000 ) ) ;
#70376=CARTESIAN_POINT ( 'NONE',  ( -0.8500000000000395017, 2.500000000000000000, 2.165063509461097713 ) ) ;
#70377=ADVANCED_FACE ( 'NONE', ( #128941 ), #14079, .T. ) ;
#70378=DIRECTION ( 'NONE',  ( 0.000000000000000000, 0.000000000000000000, 1.000000000000000000 ) ) ;
#70379=AXIS2_PLACEMENT_3D ( 'NONE', #24671, #66512, #95345 ) ;
#70380=ORIENTED_EDGE ( 'NONE', *, *, #46806, .T. ) ;
#70381=AXIS2_PLACEMENT_3D ( 'NONE', #104349, #86636, #65045 ) ;
#70382=ORIENTED_EDGE ( 'NONE', *, *, #103657, .T. ) ;
#70383=ORIENTED_EDGE ( 'NONE', *, *, #17643, .F. ) ;
#70384=CIRCLE ( 'NONE', #61983, 0.06509327318403745899 ) ;
#70385=ORIENTED_EDGE ( 'NONE', *, *, #107319, .F. ) ;
#70386=ORIENTED_EDGE ( 'NONE', *, *, #79862, .F. ) ;
#70388=DIRECTION ( 'NONE',  ( 0.000000000000000000, 0.000000000000000000, 1.000000000000000000 ) ) ;
#70389=DIRECTION ( 'NONE',  ( 0.000000000000000000, 0.000000000000000000, 1.000000000000000000 ) ) ;
#70390=VERTEX_POINT ( 'NONE', #98795 ) ;
#70391=FACE_OUTER_BOUND ( 'NONE', #15390, .T. ) ;
#70393=AXIS2_PLACEMENT_3D ( 'NONE', #109812, #100616, #19487 ) ;
#70394=AXIS2_PLACEMENT_3D ( 'NONE', #41355, #21043, #29576 ) ;
#70395=CARTESIAN_POINT ( 'NONE',  ( 6.899999999999928413, 12.50000000000000000, -3.918623584224389056 ) ) ;
#70397=FACE_OUTER_BOUND ( 'NONE', #2503, .T. ) ;
#70398=DIRECTION ( 'NONE',  ( -0.000000000000000000, -1.000000000000000000, -0.000000000000000000 ) ) ;
#70399=CIRCLE ( 'NONE', #87109, 0.06509327318403745899 ) ;
#70400=ORIENTED_EDGE ( 'NONE', *, *, #55826, .T. ) ;
#70401=DIRECTION ( 'NONE',  ( 0.000000000000000000, 0.000000000000000000, -1.000000000000000000 ) ) ;
#70402=VECTOR ( 'NONE', #77423, 1000.000000000000000 ) ;
#70403=EDGE_LOOP ( 'NONE', ( #1483, #48046, #74749, #106186 ) ) ;
#70404=EDGE_CURVE ( 'NONE', #53613, #48711, #119096, .T. ) ;
#70405=CIRCLE ( 'NONE', #45375, 0.1000000000000002554 ) ;
#70406=VERTEX_POINT ( 'NONE', #100728 ) ;
#70407=DIRECTION ( 'NONE',  ( -0.000000000000000000, -1.000000000000000000, -0.000000000000000000 ) ) ;
#70408=CARTESIAN_POINT ( 'NONE',  ( -5.850000000000022737, 2.500000000000000000, -6.595190528383302109 ) ) ;
#70409=CARTESIAN_POINT ( 'NONE',  ( -2.100000000000033396, 2.500000000000000000, -3.637306695894650055 ) ) ;
#70410=ORIENTED_EDGE ( 'NONE', *, *, #93885, .F. ) ;
#70411=ORIENTED_EDGE ( 'NONE', *, *, #31227, .F. ) ;
#70412=ADVANCED_FACE ( 'NONE', ( #41203 ), #61484, .T. ) ;
#70413=DIRECTION ( 'NONE',  ( 0.000000000000000000, -0.000000000000000000, 1.000000000000000000 ) ) ;
#70414=DIRECTION ( 'NONE',  ( -0.000000000000000000, 1.000000000000000000, -0.000000000000000000 ) ) ;
#70415=DIRECTION ( 'NONE',  ( 0.000000000000000000, 1.000000000000000000, 0.000000000000000000 ) ) ;
#70416=CARTESIAN_POINT ( 'NONE',  ( 5.799999999999934985, 2.500000000000000000, -4.430127018922202176 ) ) ;
#70417=ORIENTED_EDGE ( 'NONE', *, *, #89153, .F. ) ;
#70418=EDGE_CURVE ( 'NONE', #84654, #112423, #129050, .T. ) ;
#70419=CARTESIAN_POINT ( 'NONE',  ( -8.950000000000009948, 2.500000000000000000, -1.818653347947326138 ) ) ;
#70421=VECTOR ( 'NONE', #4352, 1000.000000000000000 ) ;
#70422=ADVANCED_FACE ( 'NONE', ( #62765 ), #64679, .T. ) ;
#70423=ORIENTED_EDGE ( 'NONE', *, *, #32132, .F. ) ;
#70424=DIRECTION ( 'NONE',  ( 0.000000000000000000, 0.000000000000000000, 1.000000000000000000 ) ) ;
#70425=ORIENTED_EDGE ( 'NONE', *, *, #123011, .F. ) ;
#70427=EDGE_CURVE ( 'NONE', #42111, #86508, #122969, .T. ) ;
#70428=DIRECTION ( 'NONE',  ( 0.000000000000000000, 0.000000000000000000, -1.000000000000000000 ) ) ;
#70429=CARTESIAN_POINT ( 'NONE',  ( 4.349999999999939249, 2.500000000000000000, 2.511473670974873507 ) ) ;
#70430=CARTESIAN_POINT ( 'NONE',  ( 11.64999999999990266, 2.500000000000000000, 2.165063509461097713 ) ) ;
#70431=VERTEX_POINT ( 'NONE', #62122 ) ;
#70432=EDGE_CURVE ( 'NONE', #22282, #121706, #63401, .T. ) ;
#70433=DIRECTION ( 'NONE',  ( 0.000000000000000000, 0.000000000000000000, 1.000000000000000000 ) ) ;
#70435=AXIS2_PLACEMENT_3D ( 'NONE', #35945, #77784, #98713 ) ;
#70436=AXIS2_PLACEMENT_3D ( 'NONE', #107662, #8151, #128616 ) ;
#70437=CARTESIAN_POINT ( 'NONE',  ( -9.200000000000006395, 2.500000000000000000, 4.230127018922196669 ) ) ;
#70438=ORIENTED_EDGE ( 'NONE', *, *, #12910, .T. ) ;
#70439=VERTEX_POINT ( 'NONE', #73223 ) ;
#70440=ORIENTED_EDGE ( 'NONE', *, *, #128813, .F. ) ;
#70441=CARTESIAN_POINT ( 'NONE',  ( -5.000000000000023093, 2.500000000000000000, 5.022947341949748790 ) ) ;
#70442=DIRECTION ( 'NONE',  ( 0.000000000000000000, -0.000000000000000000, 1.000000000000000000 ) ) ;
#70443=FACE_OUTER_BOUND ( 'NONE', #11746, .T. ) ;
#70444=CARTESIAN_POINT ( 'NONE',  ( -6.650000000000018119, 2.500000000000000000, -2.857883832488653741 ) ) ;
#70445=LINE ( 'NONE', #39725, #5203 ) ;
#70446=CIRCLE ( 'NONE', #126882, 0.06509327318403745899 ) ;
#70447=CARTESIAN_POINT ( 'NONE',  ( 9.349999999999916156, 2.500000000000000000, -2.511473670974877948 ) ) ;
#70448=CONICAL_SURFACE ( 'NONE', #80916, 0.1000000000000002554, 0.003490658503988666988 ) ;
#70449=DIRECTION ( 'NONE',  ( 0.000000000000000000, 1.000000000000000000, 0.000000000000000000 ) ) ;
#70450=CARTESIAN_POINT ( 'NONE',  ( 14.54999999999989235, 12.50000000000000000, -2.230156782645139391 ) ) ;
#70451=DIRECTION ( 'NONE',  ( 0.000000000000000000, 1.000000000000000000, 0.000000000000000000 ) ) ;
#70452=CIRCLE ( 'NONE', #95584, 0.09999999999999999167 ) ;
#70453=CONICAL_SURFACE ( 'NONE', #13995, 0.09999999999999982514, 0.003490658503988666988 ) ;
#70454=AXIS2_PLACEMENT_3D ( 'NONE', #976, #40932, #120751 ) ;
#70455=ORIENTED_EDGE ( 'NONE', *, *, #88571, .T. ) ;
#70456=DIRECTION ( 'NONE',  ( 0.000000000000000000, 0.000000000000000000, 1.000000000000000000 ) ) ;
#70457=FACE_OUTER_BOUND ( 'NONE', #66332, .T. ) ;
#70458=CARTESIAN_POINT ( 'NONE',  ( 11.84999999999990727, 2.500000000000000000, 6.148780366869520009 ) ) ;
#70459=DIRECTION ( 'NONE',  ( 0.000000000000000000, 0.000000000000000000, -1.000000000000000000 ) ) ;
#70460=ORIENTED_EDGE ( 'NONE', *, *, #128811, .F. ) ;
#70461=FACE_OUTER_BOUND ( 'NONE', #7366, .T. ) ;
#70462=ADVANCED_FACE ( 'NONE', ( #113137 ), #1564, .T. ) ;
#70464=CARTESIAN_POINT ( 'NONE',  ( -0.8000000000000376810, 12.50000000000000000, -4.265033745738164406 ) ) ;
#70465=EDGE_LOOP ( 'NONE', ( #125387, #65660 ) ) ;
#70466=CIRCLE ( 'NONE', #14016, 0.1000000000000002554 ) ;
#70467=VERTEX_POINT ( 'NONE', #84322 ) ;
#70468=AXIS2_PLACEMENT_3D ( 'NONE', #91156, #112088, #22436 ) ;
#70469=FACE_OUTER_BOUND ( 'NONE', #71580, .T. ) ;
#70471=ORIENTED_EDGE ( 'NONE', *, *, #34425, .F. ) ;
#70472=EDGE_LOOP ( 'NONE', ( #70234, #106134, #82413, #29074 ) ) ;
#70473=CARTESIAN_POINT ( 'NONE',  ( -11.25000000000000000, 2.500000000000000000, 7.088010851410848190 ) ) ;
#70474=DIRECTION ( 'NONE',  ( -0.000000000000000000, 1.000000000000000000, -0.000000000000000000 ) ) ;
#70475=DIRECTION ( 'NONE',  ( -0.000000000000000000, -1.000000000000000000, -0.000000000000000000 ) ) ;
#70476=CARTESIAN_POINT ( 'NONE',  ( -12.69999999999999218, 2.500000000000000000, -0.4464101615137741064 ) ) ;
#70477=ORIENTED_EDGE ( 'NONE', *, *, #76296, .F. ) ;
#70478=AXIS2_PLACEMENT_3D ( 'NONE', #106685, #16980, #56923 ) ;
#70479=DIRECTION ( 'NONE',  ( 0.000000000000000000, 0.000000000000000000, 1.000000000000000000 ) ) ;
#70480=ORIENTED_EDGE ( 'NONE', *, *, #96313, .T. ) ;
#70481=DIRECTION ( 'NONE',  ( 0.000000000000000000, 1.000000000000000000, 0.000000000000000000 ) ) ;
#70482=CARTESIAN_POINT ( 'NONE',  ( 17.49999999999999645, 2.413244906437269854, 3.595454705090515901 ) ) ;
#70483=AXIS2_PLACEMENT_3D ( 'NONE', #86978, #79740, #28719 ) ;
#70484=CARTESIAN_POINT ( 'NONE',  ( 17.49149623775398155, -2.500000000000000000, 4.292098716152740856 ) ) ;
#70485=ORIENTED_EDGE ( 'NONE', *, *, #71089, .F. ) ;
#70486=AXIS2_PLACEMENT_3D ( 'NONE', #43046, #23354, #33833 ) ;
#70488=EDGE_LOOP ( 'NONE', ( #102097, #50428, #2292, #35497 ) ) ;
#70489=ORIENTED_EDGE ( 'NONE', *, *, #74654, .F. ) ;
#70490=EDGE_LOOP ( 'NONE', ( #50632, #7869, #56763, #88211 ) ) ;
#70491=DIRECTION ( 'NONE',  ( 0.000000000000000000, 0.000000000000000000, 1.000000000000000000 ) ) ;
#70492=CARTESIAN_POINT ( 'NONE',  ( 8.920123399939686948, 2.500000000000000888, 8.410822907404332582 ) ) ;
#70493=DIRECTION ( 'NONE',  ( 0.000000000000000000, 0.000000000000000000, -1.000000000000000000 ) ) ;
#70494=FACE_BOUND ( 'NONE', #97114, .T. ) ;
#70495=CARTESIAN_POINT ( 'NONE',  ( -4.350000000000023626, 2.500000000000000000, 6.941600689897073018 ) ) ;
#70497=DIRECTION ( 'NONE',  ( 0.000000000000000000, 0.000000000000000000, -1.000000000000000000 ) ) ;
#70498=FACE_OUTER_BOUND ( 'NONE', #55908, .T. ) ;
#70499=DIRECTION ( 'NONE',  ( 0.000000000000000000, 0.000000000000000000, 1.000000000000000000 ) ) ;
#70500=PLANE ( 'NONE',  #107400 ) ;
#70501=VECTOR ( 'NONE', #124947, 1000.000000000000000 ) ;
#70502=DIRECTION ( 'NONE',  ( 0.000000000000000000, 0.000000000000000000, 1.000000000000000000 ) ) ;
#70503=ADVANCED_FACE ( 'NONE', ( #111863 ), #43142, .T. ) ;
#70504=DIRECTION ( 'NONE',  ( 0.000000000000000000, 1.000000000000000000, 0.000000000000000000 ) ) ;
#70505=VERTEX_POINT ( 'NONE', #102668 ) ;
#70506=ORIENTED_EDGE ( 'NONE', *, *, #72621, .F. ) ;
#70507=EDGE_LOOP ( 'NONE', ( #26155, #69850 ) ) ;
#70508=EDGE_LOOP ( 'NONE', ( #47820, #59477, #49364, #46946 ) ) ;
#70509=CARTESIAN_POINT ( 'NONE',  ( 12.04999999999990834, 12.50000000000000000, 6.495190528383297135 ) ) ;
#70510=EDGE_CURVE ( 'NONE', #7899, #62189, #89311, .T. ) ;
#70511=CARTESIAN_POINT ( 'NONE',  ( -11.89999999999999680, 2.500000000000000000, -0.4464101615137742174 ) ) ;
#70512=FACE_BOUND ( 'NONE', #62127, .T. ) ;
#70513=ADVANCED_FACE ( 'NONE', ( #82417 ), #7822, .T. ) ;
#70514=CARTESIAN_POINT ( 'NONE',  ( 1.449999999999952216, 2.500000000000000000, 1.718653347947321386 ) ) ;
#70515=AXIS2_PLACEMENT_3D ( 'NONE', #97127, #38223, #58517 ) ;
#70516=ADVANCED_FACE ( 'NONE', ( #121664 ), #35051, .T. ) ;
#70517=EDGE_CURVE ( 'NONE', #82469, #87565, #22853, .T. ) ;
#70518=VERTEX_POINT ( 'NONE', #33942 ) ;
#70519=CARTESIAN_POINT ( 'NONE',  ( -6.650000000000015454, 2.500000000000000000, 7.188010851410848723 ) ) ;
#70520=DIRECTION ( 'NONE',  ( 0.000000000000000000, 1.000000000000000000, 0.000000000000000000 ) ) ;
#70521=DIRECTION ( 'NONE',  ( 0.000000000000000000, 1.000000000000000000, 0.000000000000000000 ) ) ;
#70522=EDGE_CURVE ( 'NONE', #67262, #57482, #32025, .T. ) ;
#70523=CARTESIAN_POINT ( 'NONE',  ( 3.349999999999945466, 2.500000000000000000, -2.265063509461101798 ) ) ;
#70525=DIRECTION ( 'NONE',  ( -4.274815082592931898E-19, -0.9999939076577903929, -0.003490651415223739937 ) ) ;
#70526=AXIS2_PLACEMENT_3D ( 'NONE', #81116, #101399, #51661 ) ;
#70527=CIRCLE ( 'NONE', #51762, 0.06509327318403743123 ) ;
#70528=VERTEX_POINT ( 'NONE', #43779 ) ;
#70529=ORIENTED_EDGE ( 'NONE', *, *, #12461, .F. ) ;
#70530=DIRECTION ( 'NONE',  ( 0.000000000000000000, 1.000000000000000000, 0.000000000000000000 ) ) ;
#70531=LINE ( 'NONE', #20797, #120869 ) ;
#70532=ORIENTED_EDGE ( 'NONE', *, *, #26052, .T. ) ;
#70533=DIRECTION ( 'NONE',  ( -0.000000000000000000, 1.000000000000000000, -0.000000000000000000 ) ) ;
#70534=AXIS2_PLACEMENT_3D ( 'NONE', #107657, #12015, #70308 ) ;
#70535=AXIS2_PLACEMENT_3D ( 'NONE', #117009, #8356, #96732 ) ;
#70536=CONICAL_SURFACE ( 'NONE', #16138, 0.09999999999999982514, 0.003490658503988666988 ) ;
#70537=FACE_OUTER_BOUND ( 'NONE', #107437, .T. ) ;
#70538=DIRECTION ( 'NONE',  ( 0.000000000000000000, 0.000000000000000000, 1.000000000000000000 ) ) ;
#70539=CARTESIAN_POINT ( 'NONE',  ( 7.499999999999925393, 12.50000000000000000, -3.702399969078687292 ) ) ;
#70540=ORIENTED_EDGE ( 'NONE', *, *, #94141, .T. ) ;
#70541=DIRECTION ( 'NONE',  ( -4.274815082592931898E-19, -0.9999939076577903929, -0.003490651415223739937 ) ) ;
#70542=VERTEX_POINT ( 'NONE', #103973 ) ;
#70543=DIRECTION ( 'NONE',  ( -0.000000000000000000, -1.000000000000000000, -0.000000000000000000 ) ) ;
#70544=CIRCLE ( 'NONE', #22462, 0.1000000000000002554 ) ;
#70545=EDGE_LOOP ( 'NONE', ( #49943, #71648 ) ) ;
#70546=DIRECTION ( 'NONE',  ( 0.000000000000000000, 0.000000000000000000, -1.000000000000000000 ) ) ;
#70547=ORIENTED_EDGE ( 'NONE', *, *, #67670, .T. ) ;
#70548=DIRECTION ( 'NONE',  ( 0.000000000000000000, 1.000000000000000000, 0.000000000000000000 ) ) ;
#70549=AXIS2_PLACEMENT_3D ( 'NONE', #105661, #15964, #55902 ) ;
#70550=CARTESIAN_POINT ( 'NONE',  ( 14.14999999999989733, 2.500000000000000000, 1.472243186433545459 ) ) ;
#70551=DIRECTION ( 'NONE',  ( 0.000000000000000000, -0.000000000000000000, 1.000000000000000000 ) ) ;
#70552=DIRECTION ( 'NONE',  ( 0.000000000000000000, 0.000000000000000000, 1.000000000000000000 ) ) ;
#70553=CARTESIAN_POINT ( 'NONE',  ( -6.249999999999981348, 12.50000000000000000, 6.560283801567334372 ) ) ;
#70554=AXIS2_PLACEMENT_3D ( 'NONE', #125590, #105327, #126254 ) ;
#70555=ORIENTED_EDGE ( 'NONE', *, *, #30876, .F. ) ;
#70556=CONICAL_SURFACE ( 'NONE', #16157, 0.1000000000000002554, 0.003490658503988666988 ) ;
#70557=VERTEX_POINT ( 'NONE', #104602 ) ;
#70558=ORIENTED_EDGE ( 'NONE', *, *, #116220, .T. ) ;
#70559=DIRECTION ( 'NONE',  ( -0.000000000000000000, -1.000000000000000000, -0.000000000000000000 ) ) ;
#70560=CIRCLE ( 'NONE', #91492, 0.06509327318403745899 ) ;
#70562=CARTESIAN_POINT ( 'NONE',  ( 6.899999999999926636, 2.500000000000000000, -0.4464101615137782142 ) ) ;
#70563=EDGE_CURVE ( 'NONE', #75085, #44948, #114435, .T. ) ;
#70564=EDGE_LOOP ( 'NONE', ( #72388, #33775 ) ) ;
#70565=ORIENTED_EDGE ( 'NONE', *, *, #93965, .T. ) ;
#70566=VERTEX_POINT ( 'NONE', #91568 ) ;
#70567=EDGE_CURVE ( 'NONE', #43893, #38024, #1890, .T. ) ;
#70568=CARTESIAN_POINT ( 'NONE',  ( -10.00000000000000711, 12.50000000000000000, -3.572213422710607933 ) ) ;
#70569=CONICAL_SURFACE ( 'NONE', #41347, 0.1000000000000002554, 0.003490658503988666988 ) ;
#70571=VECTOR ( 'NONE', #11453, 1000.000000000000000 ) ;
#70572=ORIENTED_EDGE ( 'NONE', *, *, #3691, .F. ) ;
#70573=CARTESIAN_POINT ( 'NONE',  ( 7.099999999999927702, 12.50000000000000000, -3.637306695894650055 ) ) ;
#70574=AXIS2_PLACEMENT_3D ( 'NONE', #19218, #225, #80098 ) ;
#70575=CIRCLE ( 'NONE', #74788, 0.06509327318403745899 ) ;
#70576=DIRECTION ( 'NONE',  ( 0.000000000000000000, 0.000000000000000000, -1.000000000000000000 ) ) ;
#70577=DIRECTION ( 'NONE',  ( -4.274815082592931898E-19, -0.9999939076577903929, -0.003490651415223739937 ) ) ;
#70578=DIRECTION ( 'NONE',  ( 0.000000000000000000, 0.000000000000000000, 1.000000000000000000 ) ) ;
#70579=EDGE_CURVE ( 'NONE', #62109, #33637, #49623, .T. ) ;
#70580=CARTESIAN_POINT ( 'NONE',  ( 12.09999999999990195, 2.500000000000000000, 0.6928203230275494784 ) ) ;
#70581=DIRECTION ( 'NONE',  ( 0.000000000000000000, 0.000000000000000000, -1.000000000000000000 ) ) ;
#70582=EDGE_CURVE ( 'NONE', #84244, #77843, #126182, .T. ) ;
#70583=AXIS2_PLACEMENT_3D ( 'NONE', #128723, #28560, #108396 ) ;
#70584=CARTESIAN_POINT ( 'NONE',  ( 9.799999999999915445, 2.500000000000000000, -4.776537180435977525 ) ) ;
#70585=ORIENTED_EDGE ( 'NONE', *, *, #71746, .F. ) ;
#70586=EDGE_CURVE ( 'NONE', #39415, #26182, #5108, .T. ) ;
#70587=ORIENTED_EDGE ( 'NONE', *, *, #108203, .F. ) ;
#70588=LINE ( 'NONE', #95706, #23594 ) ;
#70590=CIRCLE ( 'NONE', #14131, 0.06509327318403745899 ) ;
#70591=ADVANCED_FACE ( 'NONE', ( #46327 ), #108663, .T. ) ;
#70592=DIRECTION ( 'NONE',  ( -0.000000000000000000, -1.000000000000000000, -0.000000000000000000 ) ) ;
#70593=EDGE_LOOP ( 'NONE', ( #80346, #52043 ) ) ;
#70594=ORIENTED_EDGE ( 'NONE', *, *, #95505, .T. ) ;
#70596=DIRECTION ( 'NONE',  ( 0.000000000000000000, 1.000000000000000000, 0.000000000000000000 ) ) ;
#70598=ADVANCED_FACE ( 'NONE', ( #54849 ), #97713, .T. ) ;
#70599=LINE ( 'NONE', #96994, #38508 ) ;
#70600=LINE ( 'NONE', #97476, #314 ) ;
#70601=DIRECTION ( 'NONE',  ( 0.000000000000000000, 1.000000000000000000, 0.000000000000000000 ) ) ;
#70602=CARTESIAN_POINT ( 'NONE',  ( 4.799999999999937650, 12.50000000000000000, -3.983716857408426293 ) ) ;
#70603=LINE ( 'NONE', #100067, #118760 ) ;
#70604=VECTOR ( 'NONE', #128179, 1000.000000000000000 ) ;
#70605=DIRECTION ( 'NONE',  ( 0.000000000000000000, 0.000000000000000000, -1.000000000000000000 ) ) ;
#70606=EDGE_LOOP ( 'NONE', ( #9058, #14452, #85866, #123924 ) ) ;
#70607=EDGE_LOOP ( 'NONE', ( #121584, #80165, #49389, #114068 ) ) ;
#70608=ORIENTED_EDGE ( 'NONE', *, *, #2401, .F. ) ;
#70609=EDGE_LOOP ( 'NONE', ( #87994, #38501, #125328, #7449 ) ) ;
#70610=EDGE_LOOP ( 'NONE', ( #86934, #25373, #78303, #4679 ) ) ;
#70611=CARTESIAN_POINT ( 'NONE',  ( -13.14999999999999147, 2.500000000000000000, 2.611473670974877148 ) ) ;
#70612=DIRECTION ( 'NONE',  ( -0.000000000000000000, -1.000000000000000000, -0.000000000000000000 ) ) ;
#70613=ORIENTED_EDGE ( 'NONE', *, *, #111683, .F. ) ;
#70614=AXIS2_PLACEMENT_3D ( 'NONE', #104845, #15163, #84578 ) ;
#70615=CARTESIAN_POINT ( 'NONE',  ( 3.149999999999946176, 2.500000000000000000, -1.918653347947325782 ) ) ;
#70616=VECTOR ( 'NONE', #102199, 1000.000000000000000 ) ;
#70617=DIRECTION ( 'NONE',  ( -0.000000000000000000, -1.000000000000000000, -0.000000000000000000 ) ) ;
#70618=FACE_OUTER_BOUND ( 'NONE', #71574, .T. ) ;
#70619=FACE_OUTER_BOUND ( 'NONE', #94418, .T. ) ;
#70620=ORIENTED_EDGE ( 'NONE', *, *, #116223, .F. ) ;
#70621=FACE_OUTER_BOUND ( 'NONE', #28049, .T. ) ;
#70622=AXIS2_PLACEMENT_3D ( 'NONE', #99089, #8743, #79451 ) ;
#70623=DIRECTION ( 'NONE',  ( 0.000000000000000000, 0.000000000000000000, 1.000000000000000000 ) ) ;
#70624=ORIENTED_EDGE ( 'NONE', *, *, #320, .T. ) ;
#70625=VECTOR ( 'NONE', #19037, 1000.000000000000000 ) ;
#70626=EDGE_CURVE ( 'NONE', #105627, #106720, #95440, .T. ) ;
#70627=EDGE_LOOP ( 'NONE', ( #109128, #71610 ) ) ;
#70628=VERTEX_POINT ( 'NONE', #125531 ) ;
#70629=VERTEX_POINT ( 'NONE', #75783 ) ;
#70630=DIRECTION ( 'NONE',  ( -0.000000000000000000, -1.000000000000000000, -0.000000000000000000 ) ) ;
#70631=CARTESIAN_POINT ( 'NONE',  ( 7.949999999999922018, 12.50000000000000000, -2.165063509461101710 ) ) ;
#70632=CARTESIAN_POINT ( 'NONE',  ( 15.39999999999989200, 12.50000000000000000, 0.7579135962115869374 ) ) ;
#70633=CIRCLE ( 'NONE', #116594, 0.06509327318403743123 ) ;
#70634=FACE_OUTER_BOUND ( 'NONE', #22055, .T. ) ;
#70635=ORIENTED_EDGE ( 'NONE', *, *, #36262, .T. ) ;
#70636=VECTOR ( 'NONE', #22499, 1000.000000000000000 ) ;
#70637=CARTESIAN_POINT ( 'NONE',  ( 8.749999999999918288, 2.500000000000000000, 7.088010851410848190 ) ) ;
#70638=DIRECTION ( 'NONE',  ( 0.000000000000000000, 0.000000000000000000, 1.000000000000000000 ) ) ;
#70639=CARTESIAN_POINT ( 'NONE',  ( 1.449999999999952216, 2.500000000000000000, 1.918653347947321564 ) ) ;
#70640=CARTESIAN_POINT ( 'NONE',  ( -8.749999999999976907, 12.50000000000000000, -6.495190528383297135 ) ) ;
#70642=CIRCLE ( 'NONE', #26733, 0.1000000000000002554 ) ;
#70643=DIRECTION ( 'NONE',  ( 0.000000000000000000, 0.000000000000000000, 1.000000000000000000 ) ) ;
#70644=VECTOR ( 'NONE', #61059, 1000.000000000000000 ) ;
#70645=ORIENTED_EDGE ( 'NONE', *, *, #57059, .F. ) ;
#70646=ORIENTED_EDGE ( 'NONE', *, *, #104377, .T. ) ;
#70647=FACE_OUTER_BOUND ( 'NONE', #44023, .T. ) ;
#70648=DIRECTION ( 'NONE',  ( -0.000000000000000000, -1.000000000000000000, -0.000000000000000000 ) ) ;
#70649=FACE_BOUND ( 'NONE', #38143, .T. ) ;
#70650=CIRCLE ( 'NONE', #3751, 0.06509327318403745899 ) ;
#70651=FACE_OUTER_BOUND ( 'NONE', #81652, .T. ) ;
#70652=CARTESIAN_POINT ( 'NONE',  ( -11.05000000000000071, 12.50000000000000000, 2.446380397790835826 ) ) ;
#70653=AXIS2_PLACEMENT_3D ( 'NONE', #11802, #51742, #52379 ) ;
#70654=DIRECTION ( 'NONE',  ( 0.000000000000000000, 0.000000000000000000, 1.000000000000000000 ) ) ;
#70656=FACE_OUTER_BOUND ( 'NONE', #68632, .T. ) ;
#70657=AXIS2_PLACEMENT_3D ( 'NONE', #3413, #43357, #113361 ) ;
#70658=PLANE ( 'NONE',  #57131 ) ;
#70659=CIRCLE ( 'NONE', #59942, 0.09999999999999982514 ) ;
#70660=DIRECTION ( 'NONE',  ( -0.000000000000000000, -1.000000000000000000, -0.000000000000000000 ) ) ;
#70661=VERTEX_POINT ( 'NONE', #16204 ) ;
#70662=DIRECTION ( 'NONE',  ( -4.274815082592931898E-19, -0.9999939076577903929, -0.003490651415223739937 ) ) ;
#70663=EDGE_CURVE ( 'NONE', #127904, #35498, #16834, .T. ) ;
#70664=DIRECTION ( 'NONE',  ( 0.000000000000000000, -0.9999939076577903929, 0.003490651415223739937 ) ) ;
#70665=ORIENTED_EDGE ( 'NONE', *, *, #92840, .T. ) ;
#70666=VERTEX_POINT ( 'NONE', #56769 ) ;
#70667=CARTESIAN_POINT ( 'NONE',  ( -6.050000000000017586, 2.500000000000000000, 6.148780366869520009 ) ) ;
#70668=EDGE_CURVE ( 'NONE', #102850, #49354, #103989, .T. ) ;
#70669=CARTESIAN_POINT ( 'NONE',  ( 1.249999999999952482, 12.50000000000000000, -5.802370205355749988 ) ) ;
#70670=FACE_BOUND ( 'NONE', #108850, .T. ) ;
#70671=ADVANCED_FACE ( 'NONE', ( #8971 ), #19440, .T. ) ;
#70672=DIRECTION ( 'NONE',  ( 0.000000000000000000, -0.9999939076577903929, 0.003490651415223739937 ) ) ;
#70673=AXIS2_PLACEMENT_3D ( 'NONE', #45004, #126783, #54800 ) ;
#70674=CIRCLE ( 'NONE', #87383, 0.06509327318403745899 ) ;
#70675=CARTESIAN_POINT ( 'NONE',  ( 6.649999999999930189, 12.50000000000000000, 7.188010851410848723 ) ) ;
#70676=EDGE_CURVE ( 'NONE', #32793, #45295, #101932, .T. ) ;
#70677=ADVANCED_FACE ( 'NONE', ( #68540 ), #24564, .T. ) ;
#70678=VERTEX_POINT ( 'NONE', #48265 ) ;
#70679=LINE ( 'NONE', #20938, #11103 ) ;
#70680=ADVANCED_FACE ( 'NONE', ( #50216 ), #51761, .T. ) ;
#70681=EDGE_CURVE ( 'NONE', #89857, #46113, #68465, .T. ) ;
#70682=DIRECTION ( 'NONE',  ( 0.000000000000000000, 1.000000000000000000, 0.000000000000000000 ) ) ;
#70683=EDGE_CURVE ( 'NONE', #51148, #97627, #41308, .T. ) ;
#70684=ORIENTED_EDGE ( 'NONE', *, *, #73193, .T. ) ;
#70685=DIRECTION ( 'NONE',  ( 0.000000000000000000, -0.000000000000000000, 1.000000000000000000 ) ) ;
#70686=CARTESIAN_POINT ( 'NONE',  ( 97.50000000000000000, 0.000000000000000000, 7.500000000000000000 ) ) ;
#70687=B_SPLINE_CURVE_WITH_KNOTS ( 'NONE', 3,
 ( #74318, #113594, #114238, #23935, #73650, #14722, #32486, #103777, #72396, #103125 ),
 .UNSPECIFIED., .F., .F.,
 ( 4, 2, 2, 2, 4 ),
 ( 4.270600654694601050E-17, 0.0006221151217586636060, 0.001244230243517284494, 0.001866345365275905383, 0.002488460487034526054 ),
 .UNSPECIFIED. ) ;
#70688=FACE_OUTER_BOUND ( 'NONE', #46745, .T. ) ;
#70690=EDGE_CURVE ( 'NONE', #79454, #50744, #108171, .T. ) ;
#70691=EDGE_CURVE ( 'NONE', #42905, #124494, #12028, .T. ) ;
#70692=ORIENTED_EDGE ( 'NONE', *, *, #41878, .T. ) ;
#70693=DIRECTION ( 'NONE',  ( 0.000000000000000000, 0.000000000000000000, -1.000000000000000000 ) ) ;
#70694=CARTESIAN_POINT ( 'NONE',  ( -13.94999999999998863, 12.50000000000000000, -1.818653347947323917 ) ) ;
#70695=CIRCLE ( 'NONE', #76959, 0.06509327318403745899 ) ;
#70697=ORIENTED_EDGE ( 'NONE', *, *, #113666, .T. ) ;
#70698=AXIS2_PLACEMENT_3D ( 'NONE', #74405, #105141, #106438 ) ;
#70699=ORIENTED_EDGE ( 'NONE', *, *, #79562, .T. ) ;
#70701=ORIENTED_EDGE ( 'NONE', *, *, #9699, .T. ) ;
#70702=DIRECTION ( 'NONE',  ( 0.000000000000000000, -0.9999939076577903929, 0.003490651415223739937 ) ) ;
#70703=CARTESIAN_POINT ( 'NONE',  ( 87.49999999999998579, -4.871203238224192766, 5.733266569811710234 ) ) ;
#70704=AXIS2_PLACEMENT_3D ( 'NONE', #9243, #98253, #58358 ) ;
#70705=CONICAL_SURFACE ( 'NONE', #12199, 0.1000000000000000472, 0.003490658503988666988 ) ;
#70706=FACE_OUTER_BOUND ( 'NONE', #126684, .T. ) ;
#70707=ORIENTED_EDGE ( 'NONE', *, *, #128484, .F. ) ;
#70708=DIRECTION ( 'NONE',  ( 0.000000000000000000, 0.000000000000000000, 1.000000000000000000 ) ) ;
#70709=CARTESIAN_POINT ( 'NONE',  ( 12.49999999999993605, 12.50000000000000000, -2.276824562219559311E-15 ) ) ;
#70710=LINE ( 'NONE', #100795, #50748 ) ;
#70711=DIRECTION ( 'NONE',  ( 0.000000000000000000, 1.000000000000000000, 0.000000000000000000 ) ) ;
#70712=DIRECTION ( 'NONE',  ( 0.000000000000000000, -0.000000000000000000, 1.000000000000000000 ) ) ;
#70713=DIRECTION ( 'NONE',  ( -0.000000000000000000, 1.000000000000000000, -0.000000000000000000 ) ) ;
#70714=AXIS2_PLACEMENT_3D ( 'NONE', #85620, #35884, #115719 ) ;
#70715=EDGE_LOOP ( 'NONE', ( #45479, #43859, #85980, #92580 ) ) ;
#70716=CIRCLE ( 'NONE', #114526, 0.06509327318403745899 ) ;
#70717=VERTEX_POINT ( 'NONE', #29926 ) ;
#70719=VERTEX_POINT ( 'NONE', #39762 ) ;
#70721=EDGE_LOOP ( 'NONE', ( #125482, #100003, #43375, #71709 ) ) ;
#70722=ORIENTED_EDGE ( 'NONE', *, *, #73542, .T. ) ;
#70724=ADVANCED_FACE ( 'NONE', ( #10280 ), #38466, .T. ) ;
#70725=CARTESIAN_POINT ( 'NONE',  ( 87.50000000000000000, 0.7169905660283039106, -7.500000000000000000 ) ) ;
#70726=ADVANCED_FACE ( 'NONE', ( #28637 ), #40399, .T. ) ;
#70727=CIRCLE ( 'NONE', #97907, 0.09999999999999999167 ) ;
#70728=CARTESIAN_POINT ( 'NONE',  ( -11.44999999999999751, 12.50000000000000000, 2.511473670974873507 ) ) ;
#70729=PLANE ( 'NONE',  #110362 ) ;
#70730=EDGE_CURVE ( 'NONE', #31372, #124183, #20742, .T. ) ;
#70732=CARTESIAN_POINT ( 'NONE',  ( 4.149999999999941735, 2.500000000000000000, -7.088010851410853519 ) ) ;
#70733=LINE ( 'NONE', #99563, #125350 ) ;
#70734=DIRECTION ( 'NONE',  ( -4.274815082592931898E-19, -0.9999939076577903929, -0.003490651415223739937 ) ) ;
#70735=DIRECTION ( 'NONE',  ( 0.000000000000000000, 0.000000000000000000, 1.000000000000000000 ) ) ;
#70736=VECTOR ( 'NONE', #53871, 1000.000000000000000 ) ;
#70737=CARTESIAN_POINT ( 'NONE',  ( -5.650000000000019895, 2.500000000000000000, 6.048780366869520364 ) ) ;
#70738=EDGE_CURVE ( 'NONE', #108554, #46396, #66413, .T. ) ;
#70739=DIRECTION ( 'NONE',  ( -0.000000000000000000, -1.000000000000000000, -0.000000000000000000 ) ) ;
#70740=EDGE_CURVE ( 'NONE', #44317, #94526, #114523, .T. ) ;
#70741=AXIS2_PLACEMENT_3D ( 'NONE', #52255, #60160, #121624 ) ;
#70742=ORIENTED_EDGE ( 'NONE', *, *, #2182, .F. ) ;
#70743=EDGE_CURVE ( 'NONE', #110598, #99172, #9983, .T. ) ;
#70744=CARTESIAN_POINT ( 'NONE',  ( -14.99999999999994671, 2.500000000000000000, -0.1000000000000000056 ) ) ;
#70745=ORIENTED_EDGE ( 'NONE', *, *, #67794, .F. ) ;
#70746=ORIENTED_EDGE ( 'NONE', *, *, #28755, .F. ) ;
#70747=CARTESIAN_POINT ( 'NONE',  ( -15.39999999999997904, 2.500000000000000000, -0.7928203230275518987 ) ) ;
#70748=CIRCLE ( 'NONE', #64484, 0.06509327318403745899 ) ;
#70749=DIRECTION ( 'NONE',  ( 0.000000000000000000, 0.000000000000000000, 1.000000000000000000 ) ) ;
#70750=ADVANCED_FACE ( 'NONE', ( #126617 ), #125316, .T. ) ;
#70751=DIRECTION ( 'NONE',  ( -0.000000000000000000, 1.000000000000000000, -0.000000000000000000 ) ) ;
#70752=CARTESIAN_POINT ( 'NONE',  ( 2.899999999999945732, 12.50000000000000000, -4.330127018922201643 ) ) ;
#70753=CARTESIAN_POINT ( 'NONE',  ( 11.64999999999990798, 2.500000000000000000, 7.188010851410848723 ) ) ;
#70754=FACE_OUTER_BOUND ( 'NONE', #49555, .T. ) ;
#70755=ORIENTED_EDGE ( 'NONE', *, *, #68057, .F. ) ;
#70756=CIRCLE ( 'NONE', #31068, 0.06509327318403745899 ) ;
#70757=ORIENTED_EDGE ( 'NONE', *, *, #119769, .T. ) ;
#70758=DIRECTION ( 'NONE',  ( -0.000000000000000000, -1.000000000000000000, -0.000000000000000000 ) ) ;
#70759=VERTEX_POINT ( 'NONE', #96479 ) ;
#70761=ORIENTED_EDGE ( 'NONE', *, *, #98044, .F. ) ;
#70762=AXIS2_PLACEMENT_3D ( 'NONE', #12232, #69881, #30618 ) ;
#70763=ADVANCED_FACE ( 'NONE', ( #77500 ), #16628, .T. ) ;
#70764=EDGE_LOOP ( 'NONE', ( #54094, #27278 ) ) ;
#70765=CARTESIAN_POINT ( 'NONE',  ( -3.350000000000028955, 2.500000000000000000, 7.188010851410848723 ) ) ;
#70766=CARTESIAN_POINT ( 'NONE',  ( -3.469446951953614189E-14, 12.50000000000000000, -0.6928203230275519209 ) ) ;
#70767=AXIS2_PLACEMENT_3D ( 'NONE', #96026, #37118, #25336 ) ;
#70768=CARTESIAN_POINT ( 'NONE',  ( 7.949999999999925571, 2.500000000000000000, -6.395190528383301931 ) ) ;
#70769=CARTESIAN_POINT ( 'NONE',  ( -4.350000000000027178, 12.50000000000000000, -6.841600689897077814 ) ) ;
#70770=CARTESIAN_POINT ( 'NONE',  ( 17.50000000000000000, 0.8333333333333314830, 4.000000000000000000 ) ) ;
#70771=EDGE_LOOP ( 'NONE', ( #86181, #7224, #119432, #38748 ) ) ;
#70772=DIRECTION ( 'NONE',  ( 0.000000000000000000, 1.000000000000000000, 0.000000000000000000 ) ) ;
#70773=DIRECTION ( 'NONE',  ( 0.000000000000000000, 0.000000000000000000, 1.000000000000000000 ) ) ;
#70774=DIRECTION ( 'NONE',  ( -0.000000000000000000, -1.000000000000000000, -0.000000000000000000 ) ) ;
#70775=DIRECTION ( 'NONE',  ( 0.000000000000000000, -0.000000000000000000, 1.000000000000000000 ) ) ;
#70776=PLANE ( 'NONE',  #45954 ) ;
#70777=ORIENTED_EDGE ( 'NONE', *, *, #64874, .T. ) ;
#70778=EDGE_CURVE ( 'NONE', #8819, #65023, #35652, .T. ) ;
#70779=VERTEX_POINT ( 'NONE', #25829 ) ;
#70780=CIRCLE ( 'NONE', #77048, 0.1000000000000002554 ) ;
#70781=DIRECTION ( 'NONE',  ( -0.000000000000000000, 1.000000000000000000, -0.000000000000000000 ) ) ;
#70782=ORIENTED_EDGE ( 'NONE', *, *, #116604, .F. ) ;
#70783=CARTESIAN_POINT ( 'NONE',  ( -11.64999999999999680, 12.50000000000000000, 7.122917578226811486 ) ) ;
#70785=AXIS2_PLACEMENT_3D ( 'NONE', #79950, #108756, #119877 ) ;
#70786=VECTOR ( 'NONE', #24881, 1000.000000000000000 ) ;
#70787=AXIS2_PLACEMENT_3D ( 'NONE', #90855, #1185, #41134 ) ;
#70788=ORIENTED_EDGE ( 'NONE', *, *, #48330, .F. ) ;
#70790=CARTESIAN_POINT ( 'NONE',  ( -10.60000000000000142, 12.50000000000000000, 3.918623584224383727 ) ) ;
#70792=CARTESIAN_POINT ( 'NONE',  ( 10.64999999999990976, 12.50000000000000000, 2.446380397790835826 ) ) ;
#70793=DIRECTION ( 'NONE',  ( 0.000000000000000000, 1.000000000000000000, 0.000000000000000000 ) ) ;
#70794=AXIS2_PLACEMENT_3D ( 'NONE', #102435, #94371, #122081 ) ;
#70795=CIRCLE ( 'NONE', #62503, 0.06509327318403741736 ) ;
#70796=CIRCLE ( 'NONE', #16492, 0.1000000000000002554 ) ;
#70797=FACE_OUTER_BOUND ( 'NONE', #85330, .T. ) ;
#70798=VERTEX_POINT ( 'NONE', #27750 ) ;
#70799=CARTESIAN_POINT ( 'NONE',  ( 76.40064913000593094, 3.742349286023933796, -5.987206112383456791 ) ) ;
#70800=DIRECTION ( 'NONE',  ( 0.000000000000000000, -0.000000000000000000, 1.000000000000000000 ) ) ;
#70801=CONICAL_SURFACE ( 'NONE', #91733, 0.1000000000000002554, 0.003490658503988666988 ) ;
#70802=DIRECTION ( 'NONE',  ( 0.000000000000000000, 0.000000000000000000, 1.000000000000000000 ) ) ;
#70803=DIRECTION ( 'NONE',  ( -0.000000000000000000, 1.000000000000000000, -0.000000000000000000 ) ) ;
#70804=AXIS2_PLACEMENT_3D ( 'NONE', #44523, #126315, #125648 ) ;
#70805=EDGE_LOOP ( 'NONE', ( #71244, #73921 ) ) ;
#70806=ORIENTED_EDGE ( 'NONE', *, *, #98579, .F. ) ;
#70807=CARTESIAN_POINT ( 'NONE',  ( 6.449999999999931788, 2.500000000000000000, 6.148780366869520009 ) ) ;
#70808=DIRECTION ( 'NONE',  ( 0.000000000000000000, 1.000000000000000000, 0.000000000000000000 ) ) ;
#70809=FACE_OUTER_BOUND ( 'NONE', #98068, .T. ) ;
#70810=EDGE_LOOP ( 'NONE', ( #6115, #105530 ) ) ;
#70811=AXIS2_PLACEMENT_3D ( 'NONE', #115772, #105956, #26113 ) ;
#70812=DIRECTION ( 'NONE',  ( 0.000000000000000000, 0.000000000000000000, -1.000000000000000000 ) ) ;
#70813=ADVANCED_FACE ( 'NONE', ( #36945 ), #68559, .T. ) ;
#70814=DIRECTION ( 'NONE',  ( -0.000000000000000000, -1.000000000000000000, -0.000000000000000000 ) ) ;
#70815=AXIS2_PLACEMENT_3D ( 'NONE', #66579, #95410, #37777 ) ;
#70816=ORIENTED_EDGE ( 'NONE', *, *, #18089, .F. ) ;
#70817=CARTESIAN_POINT ( 'NONE',  ( 14.14999999999989377, 2.500000000000000000, -2.957883832488653830 ) ) ;
#70819=LINE ( 'NONE', #90447, #122725 ) ;
#70820=EDGE_CURVE ( 'NONE', #115112, #18179, #38239, .T. ) ;
#70821=ORIENTED_EDGE ( 'NONE', *, *, #79299, .F. ) ;
#70822=AXIS2_PLACEMENT_3D ( 'NONE', #18751, #119525, #108420 ) ;
#70823=CARTESIAN_POINT ( 'NONE',  ( 4.349999999999941025, 2.500000000000000000, -1.818653347947326138 ) ) ;
#70824=DIRECTION ( 'NONE',  ( 0.000000000000000000, 0.000000000000000000, 1.000000000000000000 ) ) ;
#70825=EDGE_CURVE ( 'NONE', #108744, #4798, #112490, .T. ) ;
#70826=ORIENTED_EDGE ( 'NONE', *, *, #86452, .F. ) ;
#70827=EDGE_CURVE ( 'NONE', #115716, #94495, #45594, .T. ) ;
#70828=ORIENTED_EDGE ( 'NONE', *, *, #124240, .T. ) ;
#70829=ADVANCED_FACE ( 'NONE', ( #86674 ), #58117, .T. ) ;
#70830=EDGE_CURVE ( 'NONE', #76876, #92053, #5855, .T. ) ;
#70832=CARTESIAN_POINT ( 'NONE',  ( 15.39999999999989200, 12.50000000000000000, -0.7579135962115917113 ) ) ;
#70833=AXIS2_PLACEMENT_3D ( 'NONE', #37592, #127890, #46762 ) ;
#70834=VERTEX_POINT ( 'NONE', #95861 ) ;
#70835=DIRECTION ( 'NONE',  ( -4.274815082592931898E-19, -0.9999939076577903929, -0.003490651415223739937 ) ) ;
#70837=AXIS2_PLACEMENT_3D ( 'NONE', #34102, #64190, #125680 ) ;
#70838=EDGE_CURVE ( 'NONE', #53951, #53201, #95758, .T. ) ;
#70839=CARTESIAN_POINT ( 'NONE',  ( -7.050000000000016698, 2.500000000000000000, -6.395190528383301931 ) ) ;
#70840=FACE_OUTER_BOUND ( 'NONE', #11899, .T. ) ;
#70841=DIRECTION ( 'NONE',  ( -0.000000000000000000, 1.000000000000000000, -0.000000000000000000 ) ) ;
#70842=DIRECTION ( 'NONE',  ( 0.000000000000000000, 1.000000000000000000, 0.000000000000000000 ) ) ;
#70843=CARTESIAN_POINT ( 'NONE',  ( -14.59999999999998366, 2.500000000000000000, 0.7928203230275517877 ) ) ;
#70844=CIRCLE ( 'NONE', #20765, 0.1000000000000002554 ) ;
#70845=EDGE_CURVE ( 'NONE', #81499, #12633, #118740, .T. ) ;
#70846=ADVANCED_FACE ( 'NONE', ( #17934 ), #67672, .T. ) ;
#70847=EDGE_CURVE ( 'NONE', #38354, #119869, #45486, .T. ) ;
#70848=EDGE_LOOP ( 'NONE', ( #116248, #32948, #76259, #41973 ) ) ;
#70849=ORIENTED_EDGE ( 'NONE', *, *, #123275, .F. ) ;
#70850=DIRECTION ( 'NONE',  ( 0.000000000000000000, 1.000000000000000000, 0.000000000000000000 ) ) ;
#70851=CONICAL_SURFACE ( 'NONE', #20687, 0.09999999999999982514, 0.003490658503988666988 ) ;
#70852=VECTOR ( 'NONE', #84979, 1000.000000000000000 ) ;
#70853=EDGE_LOOP ( 'NONE', ( #121171, #36607 ) ) ;
#70854=DIRECTION ( 'NONE',  ( 0.000000000000000000, 0.000000000000000000, 1.000000000000000000 ) ) ;
#70855=CARTESIAN_POINT ( 'NONE',  ( 9.599999999999914380, 2.500000000000000000, 3.637306695894644726 ) ) ;
#70856=FACE_OUTER_BOUND ( 'NONE', #22535, .T. ) ;
#70857=VECTOR ( 'NONE', #109655, 1000.000000000000000 ) ;
#70858=EDGE_LOOP ( 'NONE', ( #101137, #65025 ) ) ;
#70859=EDGE_LOOP ( 'NONE', ( #118342, #3403 ) ) ;
#70860=FACE_BOUND ( 'NONE', #129501, .T. ) ;
#70861=ORIENTED_EDGE ( 'NONE', *, *, #69494, .F. ) ;
#70862=ADVANCED_FACE ( 'NONE', ( #87944 ), #3717, .T. ) ;
#70863=DIRECTION ( 'NONE',  ( 0.000000000000000000, 1.000000000000000000, 0.000000000000000000 ) ) ;
#70864=DIRECTION ( 'NONE',  ( 0.000000000000000000, 0.000000000000000000, 1.000000000000000000 ) ) ;
#70865=LINE ( 'NONE', #21109, #5313 ) ;
#70866=VECTOR ( 'NONE', #31333, 1000.000000000000000 ) ;
#70867=AXIS2_PLACEMENT_3D ( 'NONE', #90758, #79027, #41045 ) ;
#70868=DIRECTION ( 'NONE',  ( 0.000000000000000000, 1.000000000000000000, 0.000000000000000000 ) ) ;
#70870=CARTESIAN_POINT ( 'NONE',  ( -4.600000000000024514, 2.500000000000000000, 5.022947341949748790 ) ) ;
#70871=DIRECTION ( 'NONE',  ( 0.000000000000000000, 1.000000000000000000, 0.000000000000000000 ) ) ;
#70872=FACE_OUTER_BOUND ( 'NONE', #85820, .T. ) ;
#70873=CARTESIAN_POINT ( 'NONE',  ( 8.749999999999957367, 2.500000000000000000, 2.165063509461097713 ) ) ;
#70874=DIRECTION ( 'NONE',  ( 0.000000000000000000, 1.000000000000000000, 0.000000000000000000 ) ) ;
#70875=FACE_OUTER_BOUND ( 'NONE', #38547, .T. ) ;
#70876=ORIENTED_EDGE ( 'NONE', *, *, #128484, .T. ) ;
#70877=EDGE_LOOP ( 'NONE', ( #16734, #19893, #20955, #117042 ) ) ;
#70878=VERTEX_POINT ( 'NONE', #86011 ) ;
#70879=ORIENTED_EDGE ( 'NONE', *, *, #31031, .T. ) ;
#70880=DIRECTION ( 'NONE',  ( 0.000000000000000000, 0.000000000000000000, 1.000000000000000000 ) ) ;
#70881=VECTOR ( 'NONE', #69222, 1000.000000000000000 ) ;
#70882=DIRECTION ( 'NONE',  ( 0.000000000000000000, -0.9999939076577903929, 0.003490651415223739937 ) ) ;
#70883=EDGE_LOOP ( 'NONE', ( #87707, #100696, #117237, #81282 ) ) ;
#70884=VERTEX_POINT ( 'NONE', #68322 ) ;
#70885=ORIENTED_EDGE ( 'NONE', *, *, #67183, .F. ) ;
#70887=CIRCLE ( 'NONE', #1824, 0.06509327318403745899 ) ;
#70888=CIRCLE ( 'NONE', #52110, 0.06509327318403745899 ) ;
#70889=FACE_OUTER_BOUND ( 'NONE', #46904, .T. ) ;
#70890=CARTESIAN_POINT ( 'NONE',  ( 0.6499999999999561684, 2.500000000000000000, -1.818653347947325916 ) ) ;
#70891=DIRECTION ( 'NONE',  ( 0.000000000000000000, 0.000000000000000000, -1.000000000000000000 ) ) ;
#70892=CARTESIAN_POINT ( 'NONE',  ( 2.499999999999945377, 12.50000000000000000, 5.022947341949748790 ) ) ;
#70893=CARTESIAN_POINT ( 'NONE',  ( 2.500000000000002220, 2.500000000000000000, 9.000000000000003553 ) ) ;
#70894=CARTESIAN_POINT ( 'NONE',  ( -4.400000000000025224, 2.500000000000000000, 0.3464101615137735735 ) ) ;
#70896=AXIS2_PLACEMENT_3D ( 'NONE', #79482, #40859, #59858 ) ;
#70897=CIRCLE ( 'NONE', #125183, 0.06509327318403745899 ) ;
#70898=CARTESIAN_POINT ( 'NONE',  ( 2.299999999999948752, 2.500000000000000000, 0.4464101615137735513 ) ) ;
#70899=ORIENTED_EDGE ( 'NONE', *, *, #109735, .T. ) ;
#70900=EDGE_CURVE ( 'NONE', #49424, #26182, #39261, .T. ) ;
#70901=CIRCLE ( 'NONE', #98073, 0.09999999999999982514 ) ;
#70902=VERTEX_POINT ( 'NONE', #102767 ) ;
#70903=VERTEX_POINT ( 'NONE', #13092 ) ;
#70904=EDGE_CURVE ( 'NONE', #45275, #102428, #22619, .T. ) ;
#70905=DIRECTION ( 'NONE',  ( -0.000000000000000000, 1.000000000000000000, -0.000000000000000000 ) ) ;
#70906=ORIENTED_EDGE ( 'NONE', *, *, #99495, .T. ) ;
#70907=ORIENTED_EDGE ( 'NONE', *, *, #125512, .F. ) ;
#70908=ORIENTED_EDGE ( 'NONE', *, *, #86841, .T. ) ;
#70909=CIRCLE ( 'NONE', #6133, 0.1000000000000000472 ) ;
#70910=DIRECTION ( 'NONE',  ( -0.000000000000000000, -1.000000000000000000, -0.000000000000000000 ) ) ;
#70911=EDGE_CURVE ( 'NONE', #17629, #72830, #91554, .T. ) ;
#70912=CIRCLE ( 'NONE', #114805, 0.09999999999999999167 ) ;
#70913=CARTESIAN_POINT ( 'NONE',  ( -10.60000000000000320, 12.50000000000000000, -4.048810130592459089 ) ) ;
#70914=DIRECTION ( 'NONE',  ( 0.000000000000000000, -0.000000000000000000, 1.000000000000000000 ) ) ;
#70915=PLANE ( 'NONE',  #118092 ) ;
#70916=DIRECTION ( 'NONE',  ( -0.000000000000000000, -1.000000000000000000, -0.000000000000000000 ) ) ;
#70917=DIRECTION ( 'NONE',  ( 0.000000000000000000, 1.000000000000000000, 0.000000000000000000 ) ) ;
#70918=ORIENTED_EDGE ( 'NONE', *, *, #91526, .T. ) ;
#70919=DIRECTION ( 'NONE',  ( -0.000000000000000000, 1.000000000000000000, -0.000000000000000000 ) ) ;
#70920=ORIENTED_EDGE ( 'NONE', *, *, #127123, .T. ) ;
#70922=DIRECTION ( 'NONE',  ( 0.000000000000000000, 0.000000000000000000, 1.000000000000000000 ) ) ;
#70924=EDGE_LOOP ( 'NONE', ( #37444, #64651 ) ) ;
#70925=PLANE ( 'NONE',  #82299 ) ;
#70926=CARTESIAN_POINT ( 'NONE',  ( -4.400000000000028777, 2.500000000000000000, -3.983716857408426293 ) ) ;
#70927=VERTEX_POINT ( 'NONE', #62229 ) ;
#70928=FACE_OUTER_BOUND ( 'NONE', #97622, .T. ) ;
#70929=EDGE_LOOP ( 'NONE', ( #104019, #95006, #111196, #92086 ) ) ;
#70930=ORIENTED_EDGE ( 'NONE', *, *, #96224, .F. ) ;
#70931=DIRECTION ( 'NONE',  ( -0.000000000000000000, -1.000000000000000000, -0.000000000000000000 ) ) ;
#70932=LINE ( 'NONE', #101035, #9542 ) ;
#70934=CARTESIAN_POINT ( 'NONE',  ( 7.049999999999930544, 2.500000000000000000, -6.395190528383301931 ) ) ;
#70935=VECTOR ( 'NONE', #93770, 1000.000000000000000 ) ;
#70936=DIRECTION ( 'NONE',  ( -0.000000000000000000, -1.000000000000000000, -0.000000000000000000 ) ) ;
#70937=ORIENTED_EDGE ( 'NONE', *, *, #92327, .F. ) ;
#70938=DIRECTION ( 'NONE',  ( 0.000000000000000000, 0.000000000000000000, 1.000000000000000000 ) ) ;
#70939=CONICAL_SURFACE ( 'NONE', #14475, 0.1000000000000000472, 0.003490658503988666988 ) ;
#70940=EDGE_LOOP ( 'NONE', ( #48151, #62243, #74402, #108690 ) ) ;
#70941=FACE_OUTER_BOUND ( 'NONE', #20078, .T. ) ;
#70942=FACE_OUTER_BOUND ( 'NONE', #85437, .T. ) ;
#70943=CIRCLE ( 'NONE', #64675, 0.1000000000000000056 ) ;
#70944=VECTOR ( 'NONE', #56786, 1000.000000000000000 ) ;
#70945=EDGE_CURVE ( 'NONE', #124866, #24620, #120794, .T. ) ;
#70946=CIRCLE ( 'NONE', #114755, 0.06509327318403745899 ) ;
#70948=DIRECTION ( 'NONE',  ( 0.000000000000000000, 1.000000000000000000, 0.000000000000000000 ) ) ;
#70949=DIRECTION ( 'NONE',  ( 0.000000000000000000, 0.000000000000000000, 1.000000000000000000 ) ) ;
#70950=EDGE_CURVE ( 'NONE', #103996, #42757, #7916, .T. ) ;
#70951=DIRECTION ( 'NONE',  ( 0.000000000000000000, 0.000000000000000000, 1.000000000000000000 ) ) ;
#70952=FACE_OUTER_BOUND ( 'NONE', #94240, .T. ) ;
#70953=EDGE_LOOP ( 'NONE', ( #45492, #129562, #7095, #81327 ) ) ;
#70954=AXIS2_PLACEMENT_3D ( 'NONE', #27934, #67855, #98588 ) ;
#70955=AXIS2_PLACEMENT_3D ( 'NONE', #16685, #86738, #6224 ) ;
#70956=DIRECTION ( 'NONE',  ( 0.000000000000000000, 1.000000000000000000, 0.000000000000000000 ) ) ;
#70957=DIRECTION ( 'NONE',  ( 0.000000000000000000, 1.000000000000000000, 0.000000000000000000 ) ) ;
#70958=DIRECTION ( 'NONE',  ( 0.000000000000000000, 0.000000000000000000, 1.000000000000000000 ) ) ;
#70959=EDGE_CURVE ( 'NONE', #93541, #46350, #83161, .T. ) ;
#70960=ORIENTED_EDGE ( 'NONE', *, *, #3499, .T. ) ;
#70961=DIRECTION ( 'NONE',  ( 0.000000000000000000, 1.000000000000000000, 0.000000000000000000 ) ) ;
#70962=VERTEX_POINT ( 'NONE', #128573 ) ;
#70963=ORIENTED_EDGE ( 'NONE', *, *, #88125, .F. ) ;
#70964=DIRECTION ( 'NONE',  ( -0.000000000000000000, -1.000000000000000000, -0.000000000000000000 ) ) ;
#70965=AXIS2_PLACEMENT_3D ( 'NONE', #74236, #14646, #4828 ) ;
#70966=VERTEX_POINT ( 'NONE', #48701 ) ;
#70967=CARTESIAN_POINT ( 'NONE',  ( 6.849999999999930367, 12.50000000000000000, -6.841600689897078702 ) ) ;
#70968=DIRECTION ( 'NONE',  ( -0.000000000000000000, 1.000000000000000000, -0.000000000000000000 ) ) ;
#70969=DIRECTION ( 'NONE',  ( -1.000000000000000000, -0.000000000000000000, 0.000000000000000000 ) ) ;
#70970=ORIENTED_EDGE ( 'NONE', *, *, #35487, .T. ) ;
#70971=AXIS2_PLACEMENT_3D ( 'NONE', #55496, #46306, #86220 ) ;
#70972=DIRECTION ( 'NONE',  ( -0.000000000000000000, 1.000000000000000000, -0.000000000000000000 ) ) ;
#70973=AXIS2_PLACEMENT_3D ( 'NONE', #15531, #24088, #26022 ) ;
#70974=EDGE_CURVE ( 'NONE', #53869, #28525, #64356, .T. ) ;
#70975=DIRECTION ( 'NONE',  ( 0.000000000000000000, 0.000000000000000000, 1.000000000000000000 ) ) ;
#70976=CARTESIAN_POINT ( 'NONE',  ( -7.900000000000014566, 2.500000000000000000, -3.537306695894649966 ) ) ;
#70977=VECTOR ( 'NONE', #35536, 1000.000000000000000 ) ;
#70978=ORIENTED_EDGE ( 'NONE', *, *, #49464, .T. ) ;
#70979=AXIS2_PLACEMENT_3D ( 'NONE', #3142, #5050, #75096 ) ;
#70981=EDGE_CURVE ( 'NONE', #78540, #81821, #29068, .T. ) ;
#70982=CONICAL_SURFACE ( 'NONE', #8277, 0.09999999999999982514, 0.003490658503988666988 ) ;
#70983=ORIENTED_EDGE ( 'NONE', *, *, #66565, .F. ) ;
#70984=ORIENTED_EDGE ( 'NONE', *, *, #71988, .T. ) ;
#70985=CARTESIAN_POINT ( 'NONE',  ( 7.499999999999925393, 2.500000000000000000, 5.022947341949748790 ) ) ;
#70986=DIRECTION ( 'NONE',  ( 0.000000000000000000, -0.000000000000000000, 1.000000000000000000 ) ) ;
#70988=ADVANCED_FACE ( 'NONE', ( #73311 ), #35140, .T. ) ;
#70989=EDGE_CURVE ( 'NONE', #3435, #112348, #38905, .T. ) ;
#70990=FACE_BOUND ( 'NONE', #3572, .T. ) ;
#70991=ORIENTED_EDGE ( 'NONE', *, *, #43244, .F. ) ;
#70992=ADVANCED_FACE ( 'NONE', ( #89259 ), #32784, .T. ) ;
#70993=CIRCLE ( 'NONE', #35500, 0.09999999999999982514 ) ;
#70994=ADVANCED_FACE ( 'NONE', ( #22945 ), #93609, .T. ) ;
#70995=CARTESIAN_POINT ( 'NONE',  ( 7.949999999999922018, 2.500000000000000000, 6.495190528383297135 ) ) ;
#70997=ORIENTED_EDGE ( 'NONE', *, *, #95095, .T. ) ;
#70998=VECTOR ( 'NONE', #59867, 1000.000000000000000 ) ;
#70999=CARTESIAN_POINT ( 'NONE',  ( 1.049999999999953637, 2.500000000000000000, -1.818653347947326138 ) ) ;
#71000=CARTESIAN_POINT ( 'NONE',  ( 17.27572160909454624, 2.230096426605390203, 5.047229640871625733 ) ) ;
#71001=AXIS2_PLACEMENT_3D ( 'NONE', #6073, #76125, #64363 ) ;
#71002=ADVANCED_FACE ( 'NONE', ( #68970 ), #85286, .T. ) ;
#71003=DIRECTION ( 'NONE',  ( 0.000000000000000000, 0.000000000000000000, 1.000000000000000000 ) ) ;
#71004=LINE ( 'NONE', #89980, #90593 ) ;
#71005=DIRECTION ( 'NONE',  ( 0.000000000000000000, 0.000000000000000000, 1.000000000000000000 ) ) ;
#71007=CARTESIAN_POINT ( 'NONE',  ( 1.849999999999951017, 2.500000000000000000, -6.148780366869526226 ) ) ;
#71008=CARTESIAN_POINT ( 'NONE',  ( -10.00000000000000355, 2.500000000000000000, 3.637306695894644726 ) ) ;
#71009=EDGE_CURVE ( 'NONE', #129161, #53205, #121768, .T. ) ;
#71010=EDGE_CURVE ( 'NONE', #1265, #122865, #125002, .T. ) ;
#71011=ORIENTED_EDGE ( 'NONE', *, *, #41295, .T. ) ;
#71012=ORIENTED_EDGE ( 'NONE', *, *, #56774, .F. ) ;
#71013=EDGE_LOOP ( 'NONE', ( #61724, #111691 ) ) ;
#71014=EDGE_LOOP ( 'NONE', ( #71130, #110113 ) ) ;
#71015=AXIS2_PLACEMENT_3D ( 'NONE', #4063, #72187, #113376 ) ;
#71016=CARTESIAN_POINT ( 'NONE',  ( -11.84999999999999609, 2.500000000000000000, 1.918653347947321564 ) ) ;
#71017=DIRECTION ( 'NONE',  ( 0.000000000000000000, 0.000000000000000000, 1.000000000000000000 ) ) ;
#71018=EDGE_LOOP ( 'NONE', ( #125808, #17976, #73368, #111726 ) ) ;
#71019=ADVANCED_FACE ( 'NONE', ( #108880 ), #60281, .T. ) ;
#71020=FACE_BOUND ( 'NONE', #84728, .T. ) ;
#71021=EDGE_CURVE ( 'NONE', #112869, #68306, #89499, .T. ) ;
#71022=CARTESIAN_POINT ( 'NONE',  ( -10.20000000000000639, 12.50000000000000000, -3.983716857408421852 ) ) ;
#71023=CARTESIAN_POINT ( 'NONE',  ( 16.55763164795904174, 0.1615198509490234913, 6.093150836621333610 ) ) ;
#71024=FACE_OUTER_BOUND ( 'NONE', #23782, .T. ) ;
#71025=DIRECTION ( 'NONE',  ( 0.000000000000000000, 0.000000000000000000, 1.000000000000000000 ) ) ;
#71027=DIRECTION ( 'NONE',  ( 0.000000000000000000, 0.000000000000000000, 1.000000000000000000 ) ) ;
#71028=DIRECTION ( 'NONE',  ( 0.000000000000000000, -0.000000000000000000, 1.000000000000000000 ) ) ;
#71029=LINE ( 'NONE', #61205, #18330 ) ;
#71030=VERTEX_POINT ( 'NONE', #6382 ) ;
#71031=EDGE_LOOP ( 'NONE', ( #106462, #111852 ) ) ;
#71032=EDGE_LOOP ( 'NONE', ( #3909, #113623, #14104, #12112 ) ) ;
#71033=EDGE_LOOP ( 'NONE', ( #120668, #24953 ) ) ;
#71034=VERTEX_POINT ( 'NONE', #124909 ) ;
#71035=ORIENTED_EDGE ( 'NONE', *, *, #79610, .F. ) ;
#71036=DIRECTION ( 'NONE',  ( -0.000000000000000000, -1.000000000000000000, -0.000000000000000000 ) ) ;
#71037=AXIS2_PLACEMENT_3D ( 'NONE', #61411, #31310, #52224 ) ;
#71038=ORIENTED_EDGE ( 'NONE', *, *, #97204, .F. ) ;
#71039=CIRCLE ( 'NONE', #75235, 0.06509327318403745899 ) ;
#71040=CARTESIAN_POINT ( 'NONE',  ( 17.91370874550469949, 0.4812889678260096615, 4.985910759330083764 ) ) ;
#71041=AXIS2_PLACEMENT_3D ( 'NONE', #8193, #56635, #6882 ) ;
#71042=CARTESIAN_POINT ( 'NONE',  ( 16.31212831497983728, -1.499999999999935163, 6.358242018216646585 ) ) ;
#71043=DIRECTION ( 'NONE',  ( -4.274815082592931898E-19, -0.9999939076577903929, -0.003490651415223739937 ) ) ;
#71044=CARTESIAN_POINT ( 'NONE',  ( -12.69999999999999218, 12.50000000000000000, -0.2813168883297366696 ) ) ;
#71045=AXIS2_PLACEMENT_3D ( 'NONE', #71497, #39497, #20480 ) ;
#71046=ORIENTED_EDGE ( 'NONE', *, *, #109891, .F. ) ;
#71047=FACE_OUTER_BOUND ( 'NONE', #43952, .T. ) ;
#71048=AXIS2_PLACEMENT_3D ( 'NONE', #62418, #121971, #102332 ) ;
#71049=CIRCLE ( 'NONE', #102445, 0.1000000000000002554 ) ;
#71050=ORIENTED_EDGE ( 'NONE', *, *, #79539, .F. ) ;
#71051=ADVANCED_FACE ( 'NONE', ( #5121 ), #16846, .T. ) ;
#71052=ORIENTED_EDGE ( 'NONE', *, *, #54505, .F. ) ;
#71053=CARTESIAN_POINT ( 'NONE',  ( 9.799999999999913669, 2.500000000000000000, 4.676537180435972552 ) ) ;
#71054=EDGE_CURVE ( 'NONE', #88657, #110215, #127163, .T. ) ;
#71055=DIRECTION ( 'NONE',  ( -4.274815082592931898E-19, -0.9999939076577903929, -0.003490651415223739937 ) ) ;
#71056=DIRECTION ( 'NONE',  ( 0.000000000000000000, 0.000000000000000000, 1.000000000000000000 ) ) ;
#71057=VERTEX_POINT ( 'NONE', #126194 ) ;
#71058=EDGE_LOOP ( 'NONE', ( #16818, #129210 ) ) ;
#71059=DIRECTION ( 'NONE',  ( 0.000000000000000000, 1.000000000000000000, 0.000000000000000000 ) ) ;
#71060=CARTESIAN_POINT ( 'NONE',  ( -0.4000000000000396572, 12.50000000000000000, 4.265033745738159077 ) ) ;
#71061=DIRECTION ( 'NONE',  ( -0.000000000000000000, -1.000000000000000000, -0.000000000000000000 ) ) ;
#71062=LINE ( 'NONE', #21981, #123524 ) ;
#71063=ORIENTED_EDGE ( 'NONE', *, *, #67434, .F. ) ;
#71064=CARTESIAN_POINT ( 'NONE',  ( -11.89999999999999503, 12.50000000000000000, 4.676537180435972552 ) ) ;
#71065=ORIENTED_EDGE ( 'NONE', *, *, #119741, .T. ) ;
#71066=DIRECTION ( 'NONE',  ( 0.000000000000000000, 1.000000000000000000, 0.000000000000000000 ) ) ;
#71067=CONICAL_SURFACE ( 'NONE', #52191, 0.09999999999999999167, 0.003490658503988666988 ) ;
#71068=CONICAL_SURFACE ( 'NONE', #104507, 0.09999999999999982514, 0.003490658503988666988 ) ;
#71069=ORIENTED_EDGE ( 'NONE', *, *, #100070, .F. ) ;
#71070=CARTESIAN_POINT ( 'NONE',  ( 8.749999999999918288, 2.500000000000000000, 7.288010851410849256 ) ) ;
#71071=DIRECTION ( 'NONE',  ( 0.000000000000000000, 0.000000000000000000, -1.000000000000000000 ) ) ;
#71072=DIRECTION ( 'NONE',  ( -4.274815082592931898E-19, -0.9999939076577903929, -0.003490651415223739937 ) ) ;
#71073=DIRECTION ( 'NONE',  ( 0.000000000000000000, 0.000000000000000000, 1.000000000000000000 ) ) ;
#71074=ORIENTED_EDGE ( 'NONE', *, *, #71618, .T. ) ;
#71075=VECTOR ( 'NONE', #126443, 1000.000000000000000 ) ;
#71076=DIRECTION ( 'NONE',  ( 0.000000000000000000, -0.9999939076577903929, 0.003490651415223739937 ) ) ;
#71077=CARTESIAN_POINT ( 'NONE',  ( -12.09999999999999609, 2.500000000000000000, -3.737306695894647035 ) ) ;
#71079=ORIENTED_EDGE ( 'NONE', *, *, #82673, .F. ) ;
#71080=ORIENTED_EDGE ( 'NONE', *, *, #89942, .F. ) ;
#71081=CARTESIAN_POINT ( 'NONE',  ( -3.550000000000030909, 2.500000000000000000, -6.941600689897078347 ) ) ;
#71082=CARTESIAN_POINT ( 'NONE',  ( 9.549999999999918998, 2.500000000000000000, -6.395190528383301931 ) ) ;
#71083=CARTESIAN_POINT ( 'NONE',  ( 21.23528140090950700, 2.699413673072311948, 2.293764360948889802 ) ) ;
#71084=CARTESIAN_POINT ( 'NONE',  ( 6.849999999999929479, 12.50000000000000000, -1.818653347947326138 ) ) ;
#71085=AXIS2_PLACEMENT_3D ( 'NONE', #45889, #18832, #465 ) ;
#71086=DIRECTION ( 'NONE',  ( -0.000000000000000000, -1.000000000000000000, -0.000000000000000000 ) ) ;
#71087=DIRECTION ( 'NONE',  ( 0.000000000000000000, -0.9999939076577903929, 0.003490651415223739937 ) ) ;
#71088=AXIS2_PLACEMENT_3D ( 'NONE', #44716, #23785, #84633 ) ;
#71089=EDGE_CURVE ( 'NONE', #58995, #56093, #8009, .T. ) ;
#71090=CONICAL_SURFACE ( 'NONE', #20913, 0.1000000000000000472, 0.003490658503988666988 ) ;
#71091=CARTESIAN_POINT ( 'NONE',  ( -9.600000000000008527, 2.500000000000000000, -3.637306695894645614 ) ) ;
#71092=DIRECTION ( 'NONE',  ( 0.000000000000000000, 1.000000000000000000, 0.000000000000000000 ) ) ;
#71093=DIRECTION ( 'NONE',  ( -0.000000000000000000, 1.000000000000000000, -0.000000000000000000 ) ) ;
#71094=CONICAL_SURFACE ( 'NONE', #100349, 0.1000000000000002554, 0.003490658503988666988 ) ;
#71096=AXIS2_PLACEMENT_3D ( 'NONE', #87718, #96900, #77268 ) ;
#71097=FACE_OUTER_BOUND ( 'NONE', #49734, .T. ) ;
#71098=ADVANCED_FACE ( 'NONE', ( #25394 ), #56033, .T. ) ;
#71100=EDGE_CURVE ( 'NONE', #31773, #108185, #115063, .T. ) ;
#71101=CARTESIAN_POINT ( 'NONE',  ( 7.299999999999926104, 12.50000000000000000, 4.676537180435972552 ) ) ;
#71102=DIRECTION ( 'NONE',  ( 0.000000000000000000, 0.000000000000000000, -1.000000000000000000 ) ) ;
#71103=ORIENTED_EDGE ( 'NONE', *, *, #114606, .F. ) ;
#71104=DIRECTION ( 'NONE',  ( 0.000000000000000000, -0.9999939076577903929, 0.003490651415223739937 ) ) ;
#71105=DIRECTION ( 'NONE',  ( 0.000000000000000000, 0.000000000000000000, -1.000000000000000000 ) ) ;
#71106=LINE ( 'NONE', #62591, #8642 ) ;
#71107=EDGE_LOOP ( 'NONE', ( #17850, #110159, #50409, #90835 ) ) ;
#71109=ORIENTED_EDGE ( 'NONE', *, *, #71993, .F. ) ;
#71110=DIRECTION ( 'NONE',  ( -0.000000000000000000, -1.000000000000000000, -0.000000000000000000 ) ) ;
#71111=ORIENTED_EDGE ( 'NONE', *, *, #103507, .T. ) ;
#71112=ORIENTED_EDGE ( 'NONE', *, *, #86285, .T. ) ;
#71113=CARTESIAN_POINT ( 'NONE',  ( 0.1999999999999636513, 2.500000000000000000, -0.3464101615137760715 ) ) ;
#71114=CONICAL_SURFACE ( 'NONE', #14667, 0.1000000000000002554, 0.003490658503988666988 ) ;
#71115=AXIS2_PLACEMENT_3D ( 'NONE', #71871, #81043, #42410 ) ;
#71116=DIRECTION ( 'NONE',  ( -0.000000000000000000, 1.000000000000000000, -0.000000000000000000 ) ) ;
#71117=DIRECTION ( 'NONE',  ( -4.274815082592931898E-19, -0.9999939076577903929, -0.003490651415223739937 ) ) ;
#71118=DIRECTION ( 'NONE',  ( -0.000000000000000000, 1.000000000000000000, -0.000000000000000000 ) ) ;
#71119=ORIENTED_EDGE ( 'NONE', *, *, #76762, .F. ) ;
#71120=CONICAL_SURFACE ( 'NONE', #106709, 0.1000000000000002554, 0.003490658503988666988 ) ;
#71121=CIRCLE ( 'NONE', #115025, 0.1000000000000000472 ) ;
#71123=VERTEX_POINT ( 'NONE', #64054 ) ;
#71125=PLANE ( 'NONE',  #94786 ) ;
#71126=VERTEX_POINT ( 'NONE', #124267 ) ;
#71127=ADVANCED_FACE ( 'NONE', ( #95451 ), #65324, .T. ) ;
#71128=ORIENTED_EDGE ( 'NONE', *, *, #17003, .F. ) ;
#71129=ORIENTED_EDGE ( 'NONE', *, *, #38352, .F. ) ;
#71130=ORIENTED_EDGE ( 'NONE', *, *, #61256, .T. ) ;
#71131=FACE_OUTER_BOUND ( 'NONE', #42709, .T. ) ;
#71132=CARTESIAN_POINT ( 'NONE',  ( 13.80679872452938994, 2.500000000000256684, 7.946844944430235813 ) ) ;
#71133=FACE_OUTER_BOUND ( 'NONE', #88574, .T. ) ;
#71134=ADVANCED_FACE ( 'NONE', ( #26709 ), #99968, .T. ) ;
#71135=FACE_BOUND ( 'NONE', #85392, .T. ) ;
#71136=DIRECTION ( 'NONE',  ( 0.000000000000000000, 0.000000000000000000, -1.000000000000000000 ) ) ;
#71138=EDGE_CURVE ( 'NONE', #17715, #53612, #81188, .T. ) ;
#71139=DIRECTION ( 'NONE',  ( -0.000000000000000000, 1.000000000000000000, -0.000000000000000000 ) ) ;
#71140=CARTESIAN_POINT ( 'NONE',  ( -10.20000000000000284, 2.500000000000000000, -0.4464101615137782142 ) ) ;
#71141=ADVANCED_FACE ( 'NONE', ( #55530 ), #93698, .T. ) ;
#71142=DIRECTION ( 'NONE',  ( 0.000000000000000000, 0.000000000000000000, 1.000000000000000000 ) ) ;
#71143=EDGE_CURVE ( 'NONE', #37773, #72830, #4450, .T. ) ;
#71144=DIRECTION ( 'NONE',  ( -4.274815082592931898E-19, -0.9999939076577903929, -0.003490651415223739937 ) ) ;
#71145=EDGE_CURVE ( 'NONE', #105143, #109777, #56151, .T. ) ;
#71147=EDGE_CURVE ( 'NONE', #13968, #57293, #122952, .T. ) ;
#71148=CIRCLE ( 'NONE', #121324, 0.06509327318403745899 ) ;
#71149=CIRCLE ( 'NONE', #44061, 0.1000000000000002554 ) ;
#71150=CARTESIAN_POINT ( 'NONE',  ( -9.600000000000008527, 12.50000000000000000, -5.022947341949749678 ) ) ;
#71151=EDGE_CURVE ( 'NONE', #5884, #113395, #74925, .T. ) ;
#71152=ORIENTED_EDGE ( 'NONE', *, *, #49877, .F. ) ;
#71153=VERTEX_POINT ( 'NONE', #14292 ) ;
#71154=ORIENTED_EDGE ( 'NONE', *, *, #73101, .F. ) ;
#71155=EDGE_LOOP ( 'NONE', ( #103449, #45236 ) ) ;
#71156=ORIENTED_EDGE ( 'NONE', *, *, #4298, .T. ) ;
#71158=LINE ( 'NONE', #41724, #117676 ) ;
#71159=VERTEX_POINT ( 'NONE', #54238 ) ;
#71160=FACE_BOUND ( 'NONE', #6360, .T. ) ;
#71161=CIRCLE ( 'NONE', #31467, 0.06509327318403745899 ) ;
#71162=ADVANCED_FACE ( 'NONE', ( #84336 ), #41503, .T. ) ;
#71163=DIRECTION ( 'NONE',  ( 0.000000000000000000, 1.000000000000000000, 0.000000000000000000 ) ) ;
#71164=VERTEX_POINT ( 'NONE', #14913 ) ;
#71165=CARTESIAN_POINT ( 'NONE',  ( -6.700000000000019718, 2.500000000000000000, -0.1000000000000023925 ) ) ;
#71166=CARTESIAN_POINT ( 'NONE',  ( 7.899999999999924860, 12.50000000000000000, -5.022947341949754119 ) ) ;
#71167=DIRECTION ( 'NONE',  ( 0.000000000000000000, -0.000000000000000000, 1.000000000000000000 ) ) ;
#71168=CARTESIAN_POINT ( 'NONE',  ( -2.499999999999996003, 12.50000000000000000, -2.276824562219559311E-15 ) ) ;
#71169=VERTEX_POINT ( 'NONE', #54860 ) ;
#71170=CARTESIAN_POINT ( 'NONE',  ( -10.65000000000000213, 2.500000000000000000, 6.741600689897071952 ) ) ;
#71171=AXIS2_PLACEMENT_3D ( 'NONE', #114564, #15716, #24909 ) ;
#71172=AXIS2_PLACEMENT_3D ( 'NONE', #16845, #43790, #75165 ) ;
#71173=ORIENTED_EDGE ( 'NONE', *, *, #46458, .T. ) ;
#71174=ORIENTED_EDGE ( 'NONE', *, *, #77187, .F. ) ;
#71175=CARTESIAN_POINT ( 'NONE',  ( -5.200000000000025935, 12.50000000000000000, -3.983716857408426293 ) ) ;
#71176=LINE ( 'NONE', #75675, #62305 ) ;
#71177=ORIENTED_EDGE ( 'NONE', *, *, #91674, .T. ) ;
#71178=DIRECTION ( 'NONE',  ( 0.000000000000000000, 0.000000000000000000, 1.000000000000000000 ) ) ;
#71179=AXIS2_PLACEMENT_3D ( 'NONE', #117793, #28803, #78558 ) ;
#71180=CARTESIAN_POINT ( 'NONE',  ( 0.8499999999999557909, 2.500000000000000000, -6.395190528383301931 ) ) ;
#71181=DIRECTION ( 'NONE',  ( 0.000000000000000000, 1.000000000000000000, 0.000000000000000000 ) ) ;
#71183=CIRCLE ( 'NONE', #29431, 0.09999999999999982514 ) ;
#71184=CARTESIAN_POINT ( 'NONE',  ( 3.749999999999978684, 12.50000000000000000, -2.165063509461101710 ) ) ;
#71185=ORIENTED_EDGE ( 'NONE', *, *, #37876, .T. ) ;
#71186=DIRECTION ( 'NONE',  ( 0.000000000000000000, 0.000000000000000000, 1.000000000000000000 ) ) ;
#71187=ORIENTED_EDGE ( 'NONE', *, *, #22168, .T. ) ;
#71188=DIRECTION ( 'NONE',  ( -0.000000000000000000, 1.000000000000000000, -0.000000000000000000 ) ) ;
#71190=EDGE_CURVE ( 'NONE', #68306, #112869, #43545, .T. ) ;
#71191=DIRECTION ( 'NONE',  ( 0.000000000000000000, 0.000000000000000000, 1.000000000000000000 ) ) ;
#71192=EDGE_LOOP ( 'NONE', ( #117993, #56360 ) ) ;
#71193=CARTESIAN_POINT ( 'NONE',  ( 9.599999999999917932, 12.50000000000000000, -0.06509327318403970719 ) ) ;
#71194=DIRECTION ( 'NONE',  ( 0.000000000000000000, 0.000000000000000000, 1.000000000000000000 ) ) ;
#71196=CARTESIAN_POINT ( 'NONE',  ( 9.149999999999920419, 2.500000000000000000, 1.372243186433545370 ) ) ;
#71197=CARTESIAN_POINT ( 'NONE',  ( 2.699999999999945555, 2.500000000000000000, 3.883716857408420431 ) ) ;
#71198=DIRECTION ( 'NONE',  ( 0.000000000000000000, -0.9999939076577903929, 0.003490651415223739937 ) ) ;
#71199=ORIENTED_EDGE ( 'NONE', *, *, #126441, .F. ) ;
#71200=ORIENTED_EDGE ( 'NONE', *, *, #69404, .T. ) ;
#71201=EDGE_CURVE ( 'NONE', #1964, #91540, #106225, .T. ) ;
#71202=ORIENTED_EDGE ( 'NONE', *, *, #57527, .F. ) ;
#71203=FACE_OUTER_BOUND ( 'NONE', #62300, .T. ) ;
#71204=DIRECTION ( 'NONE',  ( 0.000000000000000000, 0.000000000000000000, 1.000000000000000000 ) ) ;
#71205=CIRCLE ( 'NONE', #16876, 0.06509327318403745899 ) ;
#71206=FACE_OUTER_BOUND ( 'NONE', #120953, .T. ) ;
#71207=ORIENTED_EDGE ( 'NONE', *, *, #76052, .T. ) ;
#71208=EDGE_LOOP ( 'NONE', ( #52868, #84972 ) ) ;
#71209=ORIENTED_EDGE ( 'NONE', *, *, #37876, .F. ) ;
#71210=VECTOR ( 'NONE', #102319, 1000.000000000000000 ) ;
#71211=AXIS2_PLACEMENT_3D ( 'NONE', #10817, #80246, #1028 ) ;
#71213=ORIENTED_EDGE ( 'NONE', *, *, #34484, .T. ) ;
#71214=DIRECTION ( 'NONE',  ( 0.000000000000000000, 1.000000000000000000, 0.000000000000000000 ) ) ;
#71215=DIRECTION ( 'NONE',  ( 0.000000000000000000, 0.000000000000000000, 1.000000000000000000 ) ) ;
#71216=DIRECTION ( 'NONE',  ( 0.000000000000000000, 0.000000000000000000, 1.000000000000000000 ) ) ;
#71218=DIRECTION ( 'NONE',  ( -0.000000000000000000, 1.000000000000000000, -0.000000000000000000 ) ) ;
#71219=CARTESIAN_POINT ( 'NONE',  ( 1.049999999999952083, 12.50000000000000000, 6.841600689897072485 ) ) ;
#71220=DIRECTION ( 'NONE',  ( 0.000000000000000000, 0.000000000000000000, 1.000000000000000000 ) ) ;
#71221=CONICAL_SURFACE ( 'NONE', #85873, 0.1000000000000002554, 0.003490658503988666988 ) ;
#71222=CARTESIAN_POINT ( 'NONE',  ( -2.300000000000033573, 12.50000000000000000, 0.3464101615137735735 ) ) ;
#71223=ORIENTED_EDGE ( 'NONE', *, *, #10919, .F. ) ;
#71224=LINE ( 'NONE', #103277, #19478 ) ;
#71225=CARTESIAN_POINT ( 'NONE',  ( 6.449999999999933564, 12.50000000000000000, -6.776507416713040577 ) ) ;
#71226=EDGE_LOOP ( 'NONE', ( #69302, #106797 ) ) ;
#71227=ORIENTED_EDGE ( 'NONE', *, *, #116238, .F. ) ;
#71229=DIRECTION ( 'NONE',  ( 0.000000000000000000, 1.000000000000000000, 0.000000000000000000 ) ) ;
#71230=CARTESIAN_POINT ( 'NONE',  ( -11.89999999999999680, 2.500000000000000000, 0.2464101615137776757 ) ) ;
#71231=DIRECTION ( 'NONE',  ( 0.000000000000000000, 1.000000000000000000, 0.000000000000000000 ) ) ;
#71232=DIRECTION ( 'NONE',  ( 0.000000000000000000, 1.000000000000000000, 0.000000000000000000 ) ) ;
#71233=EDGE_CURVE ( 'NONE', #64042, #39804, #108479, .T. ) ;
#71234=DIRECTION ( 'NONE',  ( 0.000000000000000000, 0.000000000000000000, 1.000000000000000000 ) ) ;
#71235=DIRECTION ( 'NONE',  ( -0.000000000000000000, -1.000000000000000000, -0.000000000000000000 ) ) ;
#71236=PLANE ( 'NONE',  #1767 ) ;
#71237=CARTESIAN_POINT ( 'NONE',  ( 2.949999999999945111, 2.500000000000000000, 2.065063509461097624 ) ) ;
#71238=CIRCLE ( 'NONE', #14772, 0.06509327318403745899 ) ;
#71239=ADVANCED_FACE ( 'NONE', ( #47639 ), #64448, .T. ) ;
#71240=ORIENTED_EDGE ( 'NONE', *, *, #94273, .T. ) ;
#71241=ORIENTED_EDGE ( 'NONE', *, *, #46752, .F. ) ;
#71242=ORIENTED_EDGE ( 'NONE', *, *, #1382, .F. ) ;
#71243=EDGE_CURVE ( 'NONE', #66158, #102525, #58218, .T. ) ;
#71244=ORIENTED_EDGE ( 'NONE', *, *, #17313, .F. ) ;
#71245=ORIENTED_EDGE ( 'NONE', *, *, #34112, .T. ) ;
#71246=EDGE_CURVE ( 'NONE', #74727, #885, #37814, .T. ) ;
#71247=CARTESIAN_POINT ( 'NONE',  ( 10.64999999999990976, 2.500000000000000000, 2.611473670974873151 ) ) ;
#71248=CARTESIAN_POINT ( 'NONE',  ( -8.950000000000006395, 12.50000000000000000, 6.776507416713035248 ) ) ;
#71249=CIRCLE ( 'NONE', #102723, 0.1000000000000002554 ) ;
#71250=ORIENTED_EDGE ( 'NONE', *, *, #4506, .F. ) ;
#71251=DIRECTION ( 'NONE',  ( 0.000000000000000000, 0.000000000000000000, 1.000000000000000000 ) ) ;
#71252=CARTESIAN_POINT ( 'NONE',  ( -8.350000000000012079, 2.500000000000000000, 2.857883832488649301 ) ) ;
#71253=EDGE_CURVE ( 'NONE', #79119, #91313, #31038, .T. ) ;
#71254=CARTESIAN_POINT ( 'NONE',  ( 10.79999999999991012, 2.500000000000000000, -4.230127018922201998 ) ) ;
#71256=ORIENTED_EDGE ( 'NONE', *, *, #121216, .F. ) ;
#71257=EDGE_CURVE ( 'NONE', #17899, #125450, #119580, .T. ) ;
#71258=DIRECTION ( 'NONE',  ( -0.000000000000000000, 1.000000000000000000, -0.000000000000000000 ) ) ;
#71259=LINE ( 'NONE', #111846, #52016 ) ;
#71260=CONICAL_SURFACE ( 'NONE', #87970, 0.1000000000000002554, 0.003490658503988666988 ) ;
#71261=VERTEX_POINT ( 'NONE', #8984 ) ;
#71262=AXIS2_PLACEMENT_3D ( 'NONE', #100586, #91423, #22702 ) ;
#71263=ORIENTED_EDGE ( 'NONE', *, *, #6056, .T. ) ;
#71264=ORIENTED_EDGE ( 'NONE', *, *, #58466, .T. ) ;
#71265=ORIENTED_EDGE ( 'NONE', *, *, #121482, .T. ) ;
#71266=DIRECTION ( 'NONE',  ( 0.000000000000000000, 1.000000000000000000, 0.000000000000000000 ) ) ;
#71267=AXIS2_PLACEMENT_3D ( 'NONE', #68555, #38485, #117635 ) ;
#71268=DIRECTION ( 'NONE',  ( 0.000000000000000000, 0.000000000000000000, 1.000000000000000000 ) ) ;
#71269=CARTESIAN_POINT ( 'NONE',  ( 9.149999999999915090, 2.500000000000000000, 6.495190528383297135 ) ) ;
#71270=ORIENTED_EDGE ( 'NONE', *, *, #128148, .T. ) ;
#71271=VECTOR ( 'NONE', #71645, 1000.000000000000000 ) ;
#71272=DIRECTION ( 'NONE',  ( 0.000000000000000000, 1.000000000000000000, 0.000000000000000000 ) ) ;
#71274=DIRECTION ( 'NONE',  ( 0.000000000000000000, -0.9999939076577903929, 0.003490651415223739937 ) ) ;
#71275=DIRECTION ( 'NONE',  ( -0.000000000000000000, 1.000000000000000000, -0.000000000000000000 ) ) ;
#71276=FACE_OUTER_BOUND ( 'NONE', #31204, .T. ) ;
#71277=DIRECTION ( 'NONE',  ( 0.000000000000000000, 0.000000000000000000, 1.000000000000000000 ) ) ;
#71278=ORIENTED_EDGE ( 'NONE', *, *, #111965, .T. ) ;
#71279=ORIENTED_EDGE ( 'NONE', *, *, #17211, .F. ) ;
#71280=ORIENTED_EDGE ( 'NONE', *, *, #76671, .T. ) ;
#71281=CARTESIAN_POINT ( 'NONE',  ( -11.69999999999999929, 2.500000000000000000, 1.734723475976807094E-15 ) ) ;
#71282=CARTESIAN_POINT ( 'NONE',  ( 13.09999999999989839, 2.500000000000000000, 0.3464101615137735735 ) ) ;
#71283=FACE_BOUND ( 'NONE', #101077, .T. ) ;
#71284=FACE_OUTER_BOUND ( 'NONE', #88622, .T. ) ;
#71285=DIRECTION ( 'NONE',  ( 0.000000000000000000, 1.000000000000000000, 0.000000000000000000 ) ) ;
#71286=EDGE_CURVE ( 'NONE', #85304, #103182, #1746, .T. ) ;
#71287=DIRECTION ( 'NONE',  ( 0.000000000000000000, 0.000000000000000000, 1.000000000000000000 ) ) ;
#71288=CIRCLE ( 'NONE', #56697, 0.1000000000000002554 ) ;
#71289=ADVANCED_FACE ( 'NONE', ( #107842 ), #28962, .T. ) ;
#71290=AXIS2_PLACEMENT_3D ( 'NONE', #58383, #98276, #88454 ) ;
#71291=EDGE_CURVE ( 'NONE', #82484, #27176, #66499, .T. ) ;
#71292=DIRECTION ( 'NONE',  ( 0.000000000000000000, -0.000000000000000000, 1.000000000000000000 ) ) ;
#71293=CONICAL_SURFACE ( 'NONE', #65016, 0.09999999999999982514, 0.003490658503988666988 ) ;
#71294=EDGE_CURVE ( 'NONE', #81079, #89242, #12212, .T. ) ;
#71295=CARTESIAN_POINT ( 'NONE',  ( 8.349999999999923261, 12.50000000000000000, 2.857883832488649301 ) ) ;
#71296=VERTEX_POINT ( 'NONE', #79668 ) ;
#71297=EDGE_CURVE ( 'NONE', #114385, #23310, #7694, .T. ) ;
#71298=FACE_OUTER_BOUND ( 'NONE', #98772, .T. ) ;
#71299=AXIS2_PLACEMENT_3D ( 'NONE', #62277, #72097, #81882 ) ;
#71300=CARTESIAN_POINT ( 'NONE',  ( 9.549999999999918998, 2.500000000000000000, 2.165063509461097713 ) ) ;
#71301=ADVANCED_FACE ( 'NONE', ( #69858 ), #112584, .T. ) ;
#71302=VERTEX_POINT ( 'NONE', #56779 ) ;
#71303=EDGE_LOOP ( 'NONE', ( #121915, #91643 ) ) ;
#71304=AXIS2_PLACEMENT_3D ( 'NONE', #109541, #86664, #27738 ) ;
#71305=DIRECTION ( 'NONE',  ( 0.000000000000000000, 0.000000000000000000, -1.000000000000000000 ) ) ;
#71306=CARTESIAN_POINT ( 'NONE',  ( 17.49862860983209600, -2.500000000000000000, 4.081131818001135336 ) ) ;
#71307=FACE_BOUND ( 'NONE', #26518, .T. ) ;
#71308=DIRECTION ( 'NONE',  ( 0.000000000000000000, 0.000000000000000000, -1.000000000000000000 ) ) ;
#71309=EDGE_CURVE ( 'NONE', #36155, #43212, #93561, .T. ) ;
#71310=EDGE_CURVE ( 'NONE', #13136, #12586, #127493, .T. ) ;
#71311=ORIENTED_EDGE ( 'NONE', *, *, #74503, .F. ) ;
#71312=LINE ( 'NONE', #40611, #19422 ) ;
#71313=DIRECTION ( 'NONE',  ( -0.000000000000000000, -1.000000000000000000, -0.000000000000000000 ) ) ;
#71314=VERTEX_POINT ( 'NONE', #78402 ) ;
#71315=CARTESIAN_POINT ( 'NONE',  ( 10.64999999999990976, 2.500000000000000000, -6.248780366869526759 ) ) ;
#71316=DIRECTION ( 'NONE',  ( 0.000000000000000000, 0.000000000000000000, 1.000000000000000000 ) ) ;
#71317=AXIS2_PLACEMENT_3D ( 'NONE', #28059, #37868, #28708 ) ;
#71318=CARTESIAN_POINT ( 'NONE',  ( -8.300000000000009592, 2.500000000000000000, 4.330127018922196314 ) ) ;
#71319=DIRECTION ( 'NONE',  ( 0.000000000000000000, 0.000000000000000000, 1.000000000000000000 ) ) ;
#71320=VECTOR ( 'NONE', #123707, 1000.000000000000000 ) ;
#71321=CONICAL_SURFACE ( 'NONE', #104764, 0.1000000000000000472, 0.003490658503988666988 ) ;
#71322=ORIENTED_EDGE ( 'NONE', *, *, #107356, .F. ) ;
#71323=CARTESIAN_POINT ( 'NONE',  ( -14.34999999999998543, 2.500000000000000000, -2.511473670974875727 ) ) ;
#71324=DIRECTION ( 'NONE',  ( 0.000000000000000000, 0.000000000000000000, -1.000000000000000000 ) ) ;
#71325=DIRECTION ( 'NONE',  ( 0.000000000000000000, -0.9999939076577903929, 0.003490651415223739937 ) ) ;
#71326=VERTEX_POINT ( 'NONE', #37185 ) ;
#71327=ORIENTED_EDGE ( 'NONE', *, *, #82245, .T. ) ;
#71328=FACE_OUTER_BOUND ( 'NONE', #75501, .T. ) ;
#71329=AXIS2_PLACEMENT_3D ( 'NONE', #95592, #26207, #66120 ) ;
#71330=VERTEX_POINT ( 'NONE', #77099 ) ;
#71331=CARTESIAN_POINT ( 'NONE',  ( -6.900000000000019007, 2.500000000000000000, -0.3464101615137783474 ) ) ;
#71332=AXIS2_PLACEMENT_3D ( 'NONE', #80428, #30042, #128900 ) ;
#71333=DIRECTION ( 'NONE',  ( 0.000000000000000000, 0.000000000000000000, 1.000000000000000000 ) ) ;
#71334=DIRECTION ( 'NONE',  ( -0.000000000000000000, 1.000000000000000000, -0.000000000000000000 ) ) ;
#71335=EDGE_LOOP ( 'NONE', ( #61849, #51057 ) ) ;
#71336=CARTESIAN_POINT ( 'NONE',  ( 0.8499999999999536815, 2.500000000000000000, 6.395190528383296602 ) ) ;
#71337=PLANE ( 'NONE',  #66482 ) ;
#71338=DIRECTION ( 'NONE',  ( -4.274815082592931898E-19, -0.9999939076577903929, -0.003490651415223739937 ) ) ;
#71339=CARTESIAN_POINT ( 'NONE',  ( 6.649999999999929301, 12.50000000000000000, 6.560283801567334372 ) ) ;
#71340=CARTESIAN_POINT ( 'NONE',  ( -6.700000000000016165, 2.500000000000000000, 4.330127018922196314 ) ) ;
#71341=PLANE ( 'NONE',  #110053 ) ;
#71342=VERTEX_POINT ( 'NONE', #116996 ) ;
#71343=CIRCLE ( 'NONE', #65079, 0.06509327318403745899 ) ;
#71344=EDGE_CURVE ( 'NONE', #86952, #14798, #37282, .T. ) ;
#71345=ORIENTED_EDGE ( 'NONE', *, *, #110312, .T. ) ;
#71346=DIRECTION ( 'NONE',  ( -0.000000000000000000, 1.000000000000000000, -0.000000000000000000 ) ) ;
#71347=ORIENTED_EDGE ( 'NONE', *, *, #22674, .F. ) ;
#71348=DIRECTION ( 'NONE',  ( 0.000000000000000000, 0.000000000000000000, -1.000000000000000000 ) ) ;
#71349=VERTEX_POINT ( 'NONE', #90773 ) ;
#71350=ORIENTED_EDGE ( 'NONE', *, *, #96267, .F. ) ;
#71351=ORIENTED_EDGE ( 'NONE', *, *, #76511, .F. ) ;
#71352=CARTESIAN_POINT ( 'NONE',  ( 13.74999999999989697, 12.50000000000000000, 2.922977105672686982 ) ) ;
#71353=AXIS2_PLACEMENT_3D ( 'NONE', #89495, #119583, #29938 ) ;
#71354=CARTESIAN_POINT ( 'NONE',  ( -9.150000000000009237, 2.500000000000000000, 1.572243186433545548 ) ) ;
#71355=CARTESIAN_POINT ( 'NONE',  ( -13.09999999999999254, 12.50000000000000000, 0.2813168883297403888 ) ) ;
#71357=DIRECTION ( 'NONE',  ( 0.000000000000000000, 1.000000000000000000, 0.000000000000000000 ) ) ;
#71358=VECTOR ( 'NONE', #79386, 1000.000000000000000 ) ;
#71359=CIRCLE ( 'NONE', #14900, 0.1000000000000002554 ) ;
#71360=DIRECTION ( 'NONE',  ( 0.000000000000000000, -0.9999939076577903929, 0.003490651415223739937 ) ) ;
#71361=CARTESIAN_POINT ( 'NONE',  ( 21.24754738303277080, -0.7337760880902354232, 4.182111650399362723 ) ) ;
#71362=DIRECTION ( 'NONE',  ( 0.000000000000000000, 0.000000000000000000, 1.000000000000000000 ) ) ;
#71363=DIRECTION ( 'NONE',  ( -0.000000000000000000, -1.000000000000000000, -0.000000000000000000 ) ) ;
#71364=CARTESIAN_POINT ( 'NONE',  ( -15.39999999999997904, 2.500000000000000000, -0.6928203230275519209 ) ) ;
#71365=ORIENTED_EDGE ( 'NONE', *, *, #106183, .F. ) ;
#71366=DIRECTION ( 'NONE',  ( 0.000000000000000000, 0.000000000000000000, 1.000000000000000000 ) ) ;
#71367=VERTEX_POINT ( 'NONE', #12205 ) ;
#71368=ORIENTED_EDGE ( 'NONE', *, *, #116654, .T. ) ;
#71369=DIRECTION ( 'NONE',  ( -0.000000000000000000, 1.000000000000000000, -0.000000000000000000 ) ) ;
#71370=CARTESIAN_POINT ( 'NONE',  ( -9.150000000000009237, 2.500000000000000000, -1.472243186433550122 ) ) ;
#71371=CARTESIAN_POINT ( 'NONE',  ( 9.799999999999913669, 2.500000000000000000, 4.676537180435972552 ) ) ;
#71372=DIRECTION ( 'NONE',  ( 0.000000000000000000, 1.000000000000000000, 0.000000000000000000 ) ) ;
#71373=CARTESIAN_POINT ( 'NONE',  ( -10.80000000000000249, 2.500000000000000000, -4.430127018922197735 ) ) ;
#71374=VECTOR ( 'NONE', #70023, 1000.000000000000000 ) ;
#71375=DIRECTION ( 'NONE',  ( 0.000000000000000000, 0.000000000000000000, 1.000000000000000000 ) ) ;
#71376=VERTEX_POINT ( 'NONE', #102527 ) ;
#71377=CONICAL_SURFACE ( 'NONE', #67242, 0.09999999999999999167, 0.003490658503988666988 ) ;
#71378=CIRCLE ( 'NONE', #83991, 0.06509327318403745899 ) ;
#71379=ORIENTED_EDGE ( 'NONE', *, *, #7684, .F. ) ;
#71380=ADVANCED_FACE ( 'NONE', ( #32529 ), #66594, .T. ) ;
#71381=VECTOR ( 'NONE', #103332, 1000.000000000000000 ) ;
#71382=ORIENTED_EDGE ( 'NONE', *, *, #2026, .F. ) ;
#71383=CONICAL_SURFACE ( 'NONE', #83914, 0.1000000000000002554, 0.003490658503988666988 ) ;
#71384=DIRECTION ( 'NONE',  ( 0.000000000000000000, 0.000000000000000000, 1.000000000000000000 ) ) ;
#71385=EDGE_LOOP ( 'NONE', ( #69304, #45495, #117282, #3595 ) ) ;
#71386=VECTOR ( 'NONE', #96468, 1000.000000000000000 ) ;
#71387=EDGE_CURVE ( 'NONE', #3248, #92137, #111710, .T. ) ;
#71388=VERTEX_POINT ( 'NONE', #121506 ) ;
#71389=ADVANCED_FACE ( 'NONE', ( #71792 ), #105232, .T. ) ;
#71391=DIRECTION ( 'NONE',  ( 0.000000000000000000, 0.000000000000000000, -1.000000000000000000 ) ) ;
#71392=CARTESIAN_POINT ( 'NONE',  ( -9.350000000000004974, 12.50000000000000000, 6.841600689897072485 ) ) ;
#71393=CARTESIAN_POINT ( 'NONE',  ( -9.600000000000008527, 2.500000000000000000, -4.230127018922197557 ) ) ;
#71394=EDGE_CURVE ( 'NONE', #2839, #51372, #72870, .T. ) ;
#71395=CARTESIAN_POINT ( 'NONE',  ( -2.100000000000033840, 2.500000000000000000, 5.022947341949748790 ) ) ;
#71396=EDGE_CURVE ( 'NONE', #74917, #118649, #95293, .T. ) ;
#71397=VERTEX_POINT ( 'NONE', #64534 ) ;
#71398=DIRECTION ( 'NONE',  ( -0.000000000000000000, -1.000000000000000000, -0.000000000000000000 ) ) ;
#71399=FACE_OUTER_BOUND ( 'NONE', #104197, .T. ) ;
#71400=ADVANCED_FACE ( 'NONE', ( #46186 ), #129421, .T. ) ;
#71401=DIRECTION ( 'NONE',  ( 0.000000000000000000, 0.000000000000000000, -1.000000000000000000 ) ) ;
#71402=EDGE_CURVE ( 'NONE', #36999, #102877, #14354, .T. ) ;
#71403=CARTESIAN_POINT ( 'NONE',  ( 6.249999999999967137, 12.50000000000000000, -2.165063509461101710 ) ) ;
#71404=DIRECTION ( 'NONE',  ( 0.000000000000000000, 0.000000000000000000, 1.000000000000000000 ) ) ;
#71405=ORIENTED_EDGE ( 'NONE', *, *, #90882, .T. ) ;
#71406=ORIENTED_EDGE ( 'NONE', *, *, #15872, .T. ) ;
#71407=ORIENTED_EDGE ( 'NONE', *, *, #70959, .F. ) ;
#71408=DIRECTION ( 'NONE',  ( 0.000000000000000000, 0.000000000000000000, 1.000000000000000000 ) ) ;
#71409=ADVANCED_FACE ( 'NONE', ( #75630 ), #114277, .T. ) ;
#71410=EDGE_LOOP ( 'NONE', ( #33210, #79400, #113683, #8380 ) ) ;
#71411=CARTESIAN_POINT ( 'NONE',  ( -12.09999999999999432, 2.500000000000000000, 4.922947341949748257 ) ) ;
#71412=AXIS2_PLACEMENT_3D ( 'NONE', #113107, #84295, #45033 ) ;
#71413=CARTESIAN_POINT ( 'NONE',  ( -9.350000000000004974, 2.500000000000000000, 6.148780366869520897 ) ) ;
#71414=AXIS2_PLACEMENT_3D ( 'NONE', #82017, #36156, #64946 ) ;
#71415=ORIENTED_EDGE ( 'NONE', *, *, #31519, .F. ) ;
#71416=LINE ( 'NONE', #39430, #114254 ) ;
#71417=DIRECTION ( 'NONE',  ( 0.000000000000000000, -0.9999939076577903929, 0.003490651415223739937 ) ) ;
#71418=DIRECTION ( 'NONE',  ( -0.000000000000000000, -1.000000000000000000, -0.000000000000000000 ) ) ;
#71419=FACE_OUTER_BOUND ( 'NONE', #121693, .T. ) ;
#71420=AXIS2_PLACEMENT_3D ( 'NONE', #58896, #38629, #109933 ) ;
#71421=AXIS2_PLACEMENT_3D ( 'NONE', #40976, #82825, #32452 ) ;
#71422=CIRCLE ( 'NONE', #48455, 0.1000000000000000472 ) ;
#71423=DIRECTION ( 'NONE',  ( -0.000000000000000000, -1.000000000000000000, -0.000000000000000000 ) ) ;
#71424=CIRCLE ( 'NONE', #34083, 0.1000000000000002554 ) ;
#71425=CIRCLE ( 'NONE', #14974, 0.06509327318403745899 ) ;
#71426=ORIENTED_EDGE ( 'NONE', *, *, #33329, .T. ) ;
#71427=ORIENTED_EDGE ( 'NONE', *, *, #12456, .F. ) ;
#71429=FACE_OUTER_BOUND ( 'NONE', #91751, .T. ) ;
#71430=LINE ( 'NONE', #70169, #42970 ) ;
#71431=AXIS2_PLACEMENT_3D ( 'NONE', #1087, #2350, #12180 ) ;
#71432=AXIS2_PLACEMENT_3D ( 'NONE', #46046, #85938, #6718 ) ;
#71433=CARTESIAN_POINT ( 'NONE',  ( 0.1999999999999627909, 2.500000000000000000, 0.4464101615137758272 ) ) ;
#71434=ORIENTED_EDGE ( 'NONE', *, *, #78524, .F. ) ;
#71435=CONICAL_SURFACE ( 'NONE', #31761, 0.1000000000000000472, 0.003490658503988666988 ) ;
#71436=CIRCLE ( 'NONE', #79860, 0.1000000000000002554 ) ;
#71437=ADVANCED_FACE ( 'NONE', ( #35727 ), #33175, .T. ) ;
#71438=EDGE_LOOP ( 'NONE', ( #57776, #3188 ) ) ;
#71439=ADVANCED_FACE ( 'NONE', ( #25907 ), #16394, .T. ) ;
#71440=DIRECTION ( 'NONE',  ( -4.274815082592931898E-19, -0.9999939076577903929, -0.003490651415223739937 ) ) ;
#71441=CARTESIAN_POINT ( 'NONE',  ( -6.071532165918824830E-15, 12.50000000000000000, -4.330127018922201643 ) ) ;
#71442=CIRCLE ( 'NONE', #119475, 0.06509327318403745899 ) ;
#71443=CARTESIAN_POINT ( 'NONE',  ( -6.700000000000019718, 12.50000000000000000, -0.06509327318403980434 ) ) ;
#71444=ADVANCED_FACE ( 'NONE', ( #73700 ), #106312, .T. ) ;
#71445=CARTESIAN_POINT ( 'NONE',  ( 12.94999999999990337, 2.500000000000000000, 2.165063509461097713 ) ) ;
#71446=EDGE_LOOP ( 'NONE', ( #74110, #46723 ) ) ;
#71447=DIRECTION ( 'NONE',  ( 0.000000000000000000, 1.000000000000000000, 0.000000000000000000 ) ) ;
#71448=EDGE_CURVE ( 'NONE', #10245, #114788, #125193, .T. ) ;
#71449=CARTESIAN_POINT ( 'NONE',  ( 4.349999999999941025, 2.500000000000000000, -1.918653347947326004 ) ) ;
#71450=CONICAL_SURFACE ( 'NONE', #75651, 0.1000000000000002554, 0.003490658503988666988 ) ;
#71451=VERTEX_POINT ( 'NONE', #63899 ) ;
#71452=DIRECTION ( 'NONE',  ( -0.000000000000000000, -1.000000000000000000, -0.000000000000000000 ) ) ;
#71453=ADVANCED_FACE ( 'NONE', ( #36389 ), #95939, .T. ) ;
#71454=ORIENTED_EDGE ( 'NONE', *, *, #100494, .T. ) ;
#71455=DIRECTION ( 'NONE',  ( 0.000000000000000000, 0.000000000000000000, 1.000000000000000000 ) ) ;
#71456=EDGE_CURVE ( 'NONE', #4651, #5028, #100061, .T. ) ;
#71457=EDGE_CURVE ( 'NONE', #109551, #114610, #12311, .T. ) ;
#71458=EDGE_LOOP ( 'NONE', ( #122901, #49977 ) ) ;
#71459=EDGE_CURVE ( 'NONE', #21383, #44658, #49895, .T. ) ;
#71460=ORIENTED_EDGE ( 'NONE', *, *, #76917, .T. ) ;
#71461=DIRECTION ( 'NONE',  ( 0.000000000000000000, 0.000000000000000000, -1.000000000000000000 ) ) ;
#71462=CARTESIAN_POINT ( 'NONE',  ( 2.500000000000002220, 2.500000000000000000, -8.999999999999998224 ) ) ;
#71464=VERTEX_POINT ( 'NONE', #94000 ) ;
#71465=PLANE ( 'NONE',  #39418 ) ;
#71466=DIRECTION ( 'NONE',  ( -4.274815082592931898E-19, -0.9999939076577903929, -0.003490651415223739937 ) ) ;
#71467=ORIENTED_EDGE ( 'NONE', *, *, #95807, .F. ) ;
#71468=EDGE_CURVE ( 'NONE', #67282, #74692, #84168, .T. ) ;
#71471=DIRECTION ( 'NONE',  ( 0.000000000000000000, -0.9999939076577903929, 0.003490651415223739937 ) ) ;
#71473=DIRECTION ( 'NONE',  ( 0.000000000000000000, 1.000000000000000000, 0.000000000000000000 ) ) ;
#71474=DIRECTION ( 'NONE',  ( 0.000000000000000000, 1.000000000000000000, 0.000000000000000000 ) ) ;
#71475=CIRCLE ( 'NONE', #121554, 0.06509327318403745899 ) ;
#71476=CIRCLE ( 'NONE', #38041, 0.06509327318403745899 ) ;
#71477=CARTESIAN_POINT ( 'NONE',  ( -14.34999999999998543, 2.500000000000000000, 2.411473670974877415 ) ) ;
#71478=CARTESIAN_POINT ( 'NONE',  ( -10.40000000000000213, 2.500000000000000000, 5.122947341949749323 ) ) ;
#71479=CIRCLE ( 'NONE', #111182, 0.09999999999999982514 ) ;
#71480=AXIS2_PLACEMENT_3D ( 'NONE', #13114, #113266, #43264 ) ;
#71481=ORIENTED_EDGE ( 'NONE', *, *, #38964, .F. ) ;
#71482=CONICAL_SURFACE ( 'NONE', #84001, 0.1000000000000000472, 0.003490658503988666988 ) ;
#71483=EDGE_LOOP ( 'NONE', ( #98367, #6575, #18282, #41112 ) ) ;
#71484=FACE_OUTER_BOUND ( 'NONE', #120646, .T. ) ;
#71485=EDGE_LOOP ( 'NONE', ( #9012, #20244 ) ) ;
#71486=CARTESIAN_POINT ( 'NONE',  ( 8.149999999999920419, 2.500000000000000000, -1.918653347947325782 ) ) ;
#71487=CARTESIAN_POINT ( 'NONE',  ( 2.699999999999946443, 2.500000000000000000, -3.983716857408426293 ) ) ;
#71488=CIRCLE ( 'NONE', #115289, 0.06509327318403745899 ) ;
#71489=CARTESIAN_POINT ( 'NONE',  ( 12.04999999999990479, 2.500000000000000000, 2.165063509461097713 ) ) ;
#71490=AXIS2_PLACEMENT_3D ( 'NONE', #116671, #6685, #125842 ) ;
#71491=ORIENTED_EDGE ( 'NONE', *, *, #55306, .F. ) ;
#71492=VERTEX_POINT ( 'NONE', #25239 ) ;
#71493=FACE_BOUND ( 'NONE', #48390, .T. ) ;
#71494=ORIENTED_EDGE ( 'NONE', *, *, #9637, .F. ) ;
#71495=ADVANCED_FACE ( 'NONE', ( #65158 ), #39544, .T. ) ;
#71496=CARTESIAN_POINT ( 'NONE',  ( -10.20000000000000639, 2.500000000000000000, -3.883716857408422207 ) ) ;
#71497=CARTESIAN_POINT ( 'NONE',  ( 8.949999999999921130, 12.50000000000000000, -6.841600689897078702 ) ) ;
#71498=CIRCLE ( 'NONE', #8691, 0.06509327318403741736 ) ;
#71499=CARTESIAN_POINT ( 'NONE',  ( 9.549999999999915445, 2.500000000000000000, 6.395190528383296602 ) ) ;
#71500=CARTESIAN_POINT ( 'NONE',  ( 11.84999999999990372, 2.500000000000000000, 1.818653347947321475 ) ) ;
#71501=CARTESIAN_POINT ( 'NONE',  ( -11.64999999999999680, 2.500000000000000000, 2.757883832488649656 ) ) ;
#71502=CARTESIAN_POINT ( 'NONE',  ( 6.849999999999929479, 12.50000000000000000, -2.576566944158915184 ) ) ;
#71503=PLANE ( 'NONE',  #62078 ) ;
#71504=DIRECTION ( 'NONE',  ( 0.000000000000000000, 0.000000000000000000, 1.000000000000000000 ) ) ;
#71505=CARTESIAN_POINT ( 'NONE',  ( 7.699999999999922018, 2.500000000000000000, 0.4464101615137735513 ) ) ;
#71506=DIRECTION ( 'NONE',  ( 0.000000000000000000, 0.000000000000000000, -1.000000000000000000 ) ) ;
#71507=CARTESIAN_POINT ( 'NONE',  ( -2.300000000000033573, 2.500000000000000000, 0.4464101615137735513 ) ) ;
#71508=ORIENTED_EDGE ( 'NONE', *, *, #17938, .F. ) ;
#71509=ORIENTED_EDGE ( 'NONE', *, *, #7664, .T. ) ;
#71510=EDGE_CURVE ( 'NONE', #13848, #50242, #29062, .T. ) ;
#71511=EDGE_LOOP ( 'NONE', ( #113473, #4684 ) ) ;
#71512=EDGE_LOOP ( 'NONE', ( #61908, #116179 ) ) ;
#71513=DIRECTION ( 'NONE',  ( -0.000000000000000000, -1.000000000000000000, -0.000000000000000000 ) ) ;
#71514=CARTESIAN_POINT ( 'NONE',  ( 4.599999999999940137, 2.500000000000000000, -4.330127018922201643 ) ) ;
#71515=ORIENTED_EDGE ( 'NONE', *, *, #71257, .F. ) ;
#71517=ORIENTED_EDGE ( 'NONE', *, *, #30639, .T. ) ;
#71518=DIRECTION ( 'NONE',  ( 0.000000000000000000, 0.000000000000000000, 1.000000000000000000 ) ) ;
#71519=AXIS2_PLACEMENT_3D ( 'NONE', #129410, #93966, #22661 ) ;
#71520=CARTESIAN_POINT ( 'NONE',  ( 9.999999999999911182, 12.50000000000000000, -3.702399969078687292 ) ) ;
#71521=DIRECTION ( 'NONE',  ( 0.000000000000000000, 1.000000000000000000, 0.000000000000000000 ) ) ;
#71522=DIRECTION ( 'NONE',  ( 0.000000000000000000, 0.000000000000000000, 1.000000000000000000 ) ) ;
#71523=PLANE ( 'NONE',  #114554 ) ;
#71524=FACE_OUTER_BOUND ( 'NONE', #18806, .T. ) ;
#71525=ADVANCED_FACE ( 'NONE', ( #97222 ), #31122, .T. ) ;
#71526=ORIENTED_EDGE ( 'NONE', *, *, #45971, .F. ) ;
#71527=AXIS2_PLACEMENT_3D ( 'NONE', #78391, #98638, #8975 ) ;
#71528=CIRCLE ( 'NONE', #67378, 0.1000000000000002554 ) ;
#71529=DIRECTION ( 'NONE',  ( -4.274815082592931898E-19, -0.9999939076577903929, -0.003490651415223739937 ) ) ;
#71530=ORIENTED_EDGE ( 'NONE', *, *, #96140, .T. ) ;
#71531=CONICAL_SURFACE ( 'NONE', #46386, 0.1000000000000002554, 0.003490658503988666988 ) ;
#71532=EDGE_LOOP ( 'NONE', ( #49286, #10336, #44806, #6935 ) ) ;
#71533=AXIS2_PLACEMENT_3D ( 'NONE', #86048, #66422, #27781 ) ;
#71534=VERTEX_POINT ( 'NONE', #18007 ) ;
#71535=PLANE ( 'NONE',  #63141 ) ;
#71536=ORIENTED_EDGE ( 'NONE', *, *, #92749, .F. ) ;
#71537=ORIENTED_EDGE ( 'NONE', *, *, #62027, .F. ) ;
#71538=EDGE_LOOP ( 'NONE', ( #20822, #27688 ) ) ;
#71539=AXIS2_PLACEMENT_3D ( 'NONE', #35401, #16998, #15737 ) ;
#71540=DIRECTION ( 'NONE',  ( 0.000000000000000000, 0.000000000000000000, 1.000000000000000000 ) ) ;
#71541=CIRCLE ( 'NONE', #75740, 0.06509327318403745899 ) ;
#71542=FACE_OUTER_BOUND ( 'NONE', #96465, .T. ) ;
#71543=DIRECTION ( 'NONE',  ( 0.000000000000000000, 0.000000000000000000, 1.000000000000000000 ) ) ;
#71544=CIRCLE ( 'NONE', #42224, 0.1000000000000002554 ) ;
#71545=CARTESIAN_POINT ( 'NONE',  ( 10.64999999999990976, 2.500000000000000000, 2.411473670974873862 ) ) ;
#71546=CONICAL_SURFACE ( 'NONE', #73679, 0.1000000000000000472, 0.003490658503988666988 ) ;
#71547=AXIS2_PLACEMENT_3D ( 'NONE', #66830, #106758, #17061 ) ;
#71548=DIRECTION ( 'NONE',  ( 0.000000000000000000, 0.000000000000000000, 1.000000000000000000 ) ) ;
#71549=CIRCLE ( 'NONE', #4621, 0.06509327318403745899 ) ;
#71550=CARTESIAN_POINT ( 'NONE',  ( -6.850000000000017408, 2.500000000000000000, -6.148780366869526226 ) ) ;
#71551=ORIENTED_EDGE ( 'NONE', *, *, #39014, .T. ) ;
#71552=CARTESIAN_POINT ( 'NONE',  ( 12.04999999999990479, 2.500000000000000000, 2.165063509461097713 ) ) ;
#71553=EDGE_CURVE ( 'NONE', #70779, #113276, #117468, .T. ) ;
#71554=VERTEX_POINT ( 'NONE', #68397 ) ;
#71555=AXIS2_PLACEMENT_3D ( 'NONE', #41249, #71990, #3246 ) ;
#71556=DIRECTION ( 'NONE',  ( -0.000000000000000000, -1.000000000000000000, -0.000000000000000000 ) ) ;
#71557=EDGE_LOOP ( 'NONE', ( #20861, #61326, #62764, #123887 ) ) ;
#71558=CARTESIAN_POINT ( 'NONE',  ( 8.149999999999920419, 2.500000000000000000, -2.511473670974877948 ) ) ;
#71559=ORIENTED_EDGE ( 'NONE', *, *, #68882, .T. ) ;
#71560=EDGE_CURVE ( 'NONE', #83874, #91821, #112668, .T. ) ;
#71561=CARTESIAN_POINT ( 'NONE',  ( -12.29999999999999538, 2.500000000000000000, -0.4464101615137742174 ) ) ;
#71562=FACE_OUTER_BOUND ( 'NONE', #84379, .T. ) ;
#71563=ORIENTED_EDGE ( 'NONE', *, *, #128595, .F. ) ;
#71564=EDGE_CURVE ( 'NONE', #125928, #60150, #86751, .T. ) ;
#71565=EDGE_CURVE ( 'NONE', #35564, #78919, #43637, .T. ) ;
#71566=VERTEX_POINT ( 'NONE', #69039 ) ;
#71567=CARTESIAN_POINT ( 'NONE',  ( 11.24999999999990763, 12.50000000000000000, 1.472243186433545459 ) ) ;
#71568=DIRECTION ( 'NONE',  ( 0.000000000000000000, 0.000000000000000000, 1.000000000000000000 ) ) ;
#71569=EDGE_CURVE ( 'NONE', #37534, #114066, #96557, .T. ) ;
#71571=ADVANCED_FACE ( 'NONE', ( #126688 ), #3900, .T. ) ;
#71572=CARTESIAN_POINT ( 'NONE',  ( 11.44999999999990514, 12.50000000000000000, -6.083687093685488989 ) ) ;
#71573=CARTESIAN_POINT ( 'NONE',  ( 10.64999999999991331, 12.50000000000000000, 6.148780366869520897 ) ) ;
#71574=EDGE_LOOP ( 'NONE', ( #76569, #99794, #27760, #30270 ) ) ;
#71575=CARTESIAN_POINT ( 'NONE',  ( 2.500000000000002220, -1.761799387799148686, 10.00000000000000000 ) ) ;
#71576=VECTOR ( 'NONE', #97232, 1000.000000000000000 ) ;
#71577=AXIS2_PLACEMENT_3D ( 'NONE', #118837, #27632, #106223 ) ;
#71578=CIRCLE ( 'NONE', #73712, 0.06509327318403745899 ) ;
#71579=EDGE_CURVE ( 'NONE', #62336, #119953, #20647, .T. ) ;
#71580=EDGE_LOOP ( 'NONE', ( #26446, #101810, #68782, #45470 ) ) ;
#71581=ADVANCED_FACE ( 'NONE', ( #27827 ), #66465, .T. ) ;
#71582=CARTESIAN_POINT ( 'NONE',  ( 13.74999999999989519, 12.50000000000000000, -2.792790559304616504 ) ) ;
#71584=CIRCLE ( 'NONE', #6798, 0.06509327318403745899 ) ;
#71585=ADVANCED_FACE ( 'NONE', ( #38312 ), #54084, .T. ) ;
#71587=AXIS2_PLACEMENT_3D ( 'NONE', #38724, #128387, #118529 ) ;
#71588=CIRCLE ( 'NONE', #86236, 0.1000000000000002554 ) ;
#71589=AXIS2_PLACEMENT_3D ( 'NONE', #9071, #88930, #128882 ) ;
#71591=CARTESIAN_POINT ( 'NONE',  ( 2.099999999999949463, 12.50000000000000000, 0.6277270498435120194 ) ) ;
#71592=PLANE ( 'NONE',  #17291 ) ;
#71593=DIRECTION ( 'NONE',  ( 0.000000000000000000, 0.000000000000000000, -1.000000000000000000 ) ) ;
#71594=FACE_OUTER_BOUND ( 'NONE', #5440, .T. ) ;
#71595=ORIENTED_EDGE ( 'NONE', *, *, #3748, .F. ) ;
#71596=CIRCLE ( 'NONE', #36008, 0.1000000000000000472 ) ;
#71597=DIRECTION ( 'NONE',  ( 0.000000000000000000, 0.000000000000000000, 1.000000000000000000 ) ) ;
#71598=DIRECTION ( 'NONE',  ( 0.000000000000000000, 1.000000000000000000, 0.000000000000000000 ) ) ;
#71599=DIRECTION ( 'NONE',  ( 0.000000000000000000, 1.000000000000000000, 0.000000000000000000 ) ) ;
#71600=VERTEX_POINT ( 'NONE', #106392 ) ;
#71601=CARTESIAN_POINT ( 'NONE',  ( -12.89999999999999147, 2.500000000000000000, 4.430127018922196847 ) ) ;
#71602=VERTEX_POINT ( 'NONE', #56628 ) ;
#71603=VERTEX_POINT ( 'NONE', #28490 ) ;
#71604=CARTESIAN_POINT ( 'NONE',  ( -1.900000000000034106, 2.500000000000000000, -3.983716857408426293 ) ) ;
#71605=ORIENTED_EDGE ( 'NONE', *, *, #117361, .T. ) ;
#71606=CARTESIAN_POINT ( 'NONE',  ( 19.61395058415432402, -2.556813634647812084, -4.305699210822446332 ) ) ;
#71607=CARTESIAN_POINT ( 'NONE',  ( -0.4000000000000396572, 12.50000000000000000, 4.395220292106234439 ) ) ;
#71608=CARTESIAN_POINT ( 'NONE',  ( 16.79927703354126933, 2.472530191752442263, 3.248144252800958309 ) ) ;
#71609=VECTOR ( 'NONE', #19926, 1000.000000000000000 ) ;
#71610=ORIENTED_EDGE ( 'NONE', *, *, #45144, .T. ) ;
#71611=AXIS2_PLACEMENT_3D ( 'NONE', #45907, #106739, #75346 ) ;
#71612=DIRECTION ( 'NONE',  ( 0.000000000000000000, 1.000000000000000000, 0.000000000000000000 ) ) ;
#71613=CARTESIAN_POINT ( 'NONE',  ( -13.34999999999999076, 2.500000000000000000, 2.165063509461101265 ) ) ;
#71614=EDGE_CURVE ( 'NONE', #48774, #4494, #7539, .T. ) ;
#71615=VECTOR ( 'NONE', #118783, 1000.000000000000000 ) ;
#71616=ORIENTED_EDGE ( 'NONE', *, *, #65797, .F. ) ;
#71617=CIRCLE ( 'NONE', #59016, 0.06509327318403745899 ) ;
#71618=EDGE_CURVE ( 'NONE', #102929, #2990, #104262, .T. ) ;
#71619=CIRCLE ( 'NONE', #121787, 0.1000000000000002554 ) ;
#71620=AXIS2_PLACEMENT_3D ( 'NONE', #127926, #108282, #6198 ) ;
#71621=ORIENTED_EDGE ( 'NONE', *, *, #60526, .T. ) ;
#71622=ADVANCED_FACE ( 'NONE', ( #47481 ), #70801, .T. ) ;
#71623=EDGE_LOOP ( 'NONE', ( #32291, #24159 ) ) ;
#71624=DIRECTION ( 'NONE',  ( 0.000000000000000000, -0.000000000000000000, 1.000000000000000000 ) ) ;
#71625=PLANE ( 'NONE',  #47931 ) ;
#71626=DIRECTION ( 'NONE',  ( 0.000000000000000000, 1.000000000000000000, 0.000000000000000000 ) ) ;
#71627=FACE_BOUND ( 'NONE', #120733, .T. ) ;
#71628=VERTEX_POINT ( 'NONE', #116204 ) ;
#71629=DIRECTION ( 'NONE',  ( -0.000000000000000000, 1.000000000000000000, -0.000000000000000000 ) ) ;
#71631=CONICAL_SURFACE ( 'NONE', #98815, 0.1000000000000002554, 0.003490658503988666988 ) ;
#71632=ORIENTED_EDGE ( 'NONE', *, *, #127579, .T. ) ;
#71633=EDGE_CURVE ( 'NONE', #55439, #128871, #127256, .T. ) ;
#71634=CONICAL_SURFACE ( 'NONE', #25450, 0.1000000000000002554, 0.003490658503988666988 ) ;
#71635=DIRECTION ( 'NONE',  ( 0.000000000000000000, 0.000000000000000000, 1.000000000000000000 ) ) ;
#71636=LINE ( 'NONE', #122669, #97229 ) ;
#71637=AXIS2_PLACEMENT_3D ( 'NONE', #102131, #101491, #104061 ) ;
#71638=CIRCLE ( 'NONE', #88339, 0.09999999999999982514 ) ;
#71639=CIRCLE ( 'NONE', #113409, 0.1000000000000002554 ) ;
#71640=DIRECTION ( 'NONE',  ( 0.000000000000000000, 0.000000000000000000, 1.000000000000000000 ) ) ;
#71641=CARTESIAN_POINT ( 'NONE',  ( 2.500000000000002220, 1.499999999999999334, 10.00000000000000178 ) ) ;
#71643=DIRECTION ( 'NONE',  ( 0.000000000000000000, -0.000000000000000000, 1.000000000000000000 ) ) ;
#71644=CIRCLE ( 'NONE', #529, 0.06509327318403745899 ) ;
#71645=DIRECTION ( 'NONE',  ( 0.000000000000000000, -0.9999939076577903929, 0.003490651415223739937 ) ) ;
#71646=VERTEX_POINT ( 'NONE', #87387 ) ;
#71647=CONICAL_SURFACE ( 'NONE', #67513, 0.1000000000000002554, 0.003490658503988666988 ) ;
#71648=ORIENTED_EDGE ( 'NONE', *, *, #6500, .F. ) ;
#71649=ORIENTED_EDGE ( 'NONE', *, *, #58402, .T. ) ;
#71650=EDGE_LOOP ( 'NONE', ( #44173, #38478, #86503, #66937 ) ) ;
#71651=CARTESIAN_POINT ( 'NONE',  ( 4.999999999999936939, 12.50000000000000000, -3.637306695894650055 ) ) ;
#71653=EDGE_LOOP ( 'NONE', ( #78629, #33809 ) ) ;
#71654=FACE_BOUND ( 'NONE', #109393, .T. ) ;
#71655=EDGE_CURVE ( 'NONE', #51914, #56997, #88016, .T. ) ;
#71656=CARTESIAN_POINT ( 'NONE',  ( -13.34999999999999076, 2.500000000000000000, 1.572243186433549544 ) ) ;
#71657=CARTESIAN_POINT ( 'NONE',  ( -9.800000000000006040, 2.500000000000000000, 4.676537180435972552 ) ) ;
#71658=DIRECTION ( 'NONE',  ( 0.000000000000000000, 1.000000000000000000, 0.000000000000000000 ) ) ;
#71659=CARTESIAN_POINT ( 'NONE',  ( 9.599999999999917932, 2.500000000000000000, 0.6928203230275494784 ) ) ;
#71660=CARTESIAN_POINT ( 'NONE',  ( -10.65000000000000213, 2.500000000000000000, 1.718653347947321386 ) ) ;
#71661=FACE_OUTER_BOUND ( 'NONE', #113439, .T. ) ;
#71662=DIRECTION ( 'NONE',  ( 0.000000000000000000, 1.000000000000000000, 0.000000000000000000 ) ) ;
#71663=DIRECTION ( 'NONE',  ( 0.000000000000000000, 1.000000000000000000, 0.000000000000000000 ) ) ;
#71664=DIRECTION ( 'NONE',  ( 0.000000000000000000, 1.000000000000000000, 0.000000000000000000 ) ) ;
#71665=ORIENTED_EDGE ( 'NONE', *, *, #70432, .T. ) ;
#71666=EDGE_LOOP ( 'NONE', ( #109929, #106188, #24460, #111725 ) ) ;
#71667=VERTEX_POINT ( 'NONE', #1585 ) ;
#71668=ORIENTED_EDGE ( 'NONE', *, *, #58465, .F. ) ;
#71669=EDGE_CURVE ( 'NONE', #62648, #125139, #112199, .T. ) ;
#71671=VECTOR ( 'NONE', #37680, 1000.000000000000000 ) ;
#71672=ORIENTED_EDGE ( 'NONE', *, *, #41872, .T. ) ;
#71673=CONICAL_SURFACE ( 'NONE', #15210, 0.1000000000000000472, 0.003490658503988666988 ) ;
#71674=DIRECTION ( 'NONE',  ( 0.000000000000000000, 0.000000000000000000, 1.000000000000000000 ) ) ;
#71675=EDGE_LOOP ( 'NONE', ( #77608, #102048 ) ) ;
#71676=ORIENTED_EDGE ( 'NONE', *, *, #95623, .T. ) ;
#71677=CIRCLE ( 'NONE', #126040, 0.06509327318403745899 ) ;
#71678=CONICAL_SURFACE ( 'NONE', #38243, 0.1000000000000002554, 0.003490658503988666988 ) ;
#71679=AXIS2_PLACEMENT_3D ( 'NONE', #48085, #8136, #97814 ) ;
#71680=DIRECTION ( 'NONE',  ( -0.000000000000000000, 1.000000000000000000, -0.000000000000000000 ) ) ;
#71681=CARTESIAN_POINT ( 'NONE',  ( 15.83209681635537258, -2.499999999999999556, 5.404881881984330505 ) ) ;
#71682=DIRECTION ( 'NONE',  ( 0.000000000000000000, -0.000000000000000000, 1.000000000000000000 ) ) ;
#71683=FACE_OUTER_BOUND ( 'NONE', #49361, .T. ) ;
#71684=AXIS2_PLACEMENT_3D ( 'NONE', #96146, #36612, #95509 ) ;
#71685=AXIS2_PLACEMENT_3D ( 'NONE', #100452, #9498, #30448 ) ;
#71686=EDGE_CURVE ( 'NONE', #56285, #84308, #121074, .T. ) ;
#71687=EDGE_LOOP ( 'NONE', ( #30483, #43408, #87997, #43760 ) ) ;
#71688=DIRECTION ( 'NONE',  ( -0.000000000000000000, 1.000000000000000000, -0.000000000000000000 ) ) ;
#71689=AXIS2_PLACEMENT_3D ( 'NONE', #67858, #107790, #18110 ) ;
#71691=ORIENTED_EDGE ( 'NONE', *, *, #78684, .F. ) ;
#71692=CARTESIAN_POINT ( 'NONE',  ( -5.000000000000022204, 2.500000000000000000, -0.5928203230275541635 ) ) ;
#71693=CARTESIAN_POINT ( 'NONE',  ( -10.00000000000000533, 2.500000000000000000, 0.5928203230275495006 ) ) ;
#71694=DIRECTION ( 'NONE',  ( 0.000000000000000000, 0.000000000000000000, 1.000000000000000000 ) ) ;
#71696=ORIENTED_EDGE ( 'NONE', *, *, #33764, .T. ) ;
#71697=ORIENTED_EDGE ( 'NONE', *, *, #107753, .F. ) ;
#71698=AXIS2_PLACEMENT_3D ( 'NONE', #79509, #121349, #70328 ) ;
#71699=FACE_OUTER_BOUND ( 'NONE', #72763, .T. ) ;
#71700=DIRECTION ( 'NONE',  ( -0.000000000000000000, 1.000000000000000000, -0.000000000000000000 ) ) ;
#71701=DIRECTION ( 'NONE',  ( -0.000000000000000000, 1.000000000000000000, -0.000000000000000000 ) ) ;
#71702=DIRECTION ( 'NONE',  ( 0.000000000000000000, 0.000000000000000000, -1.000000000000000000 ) ) ;
#71703=ORIENTED_EDGE ( 'NONE', *, *, #19648, .F. ) ;
#71704=CARTESIAN_POINT ( 'NONE',  ( 13.74999999999989519, 2.500000000000000000, -2.757883832488654097 ) ) ;
#71705=AXIS2_PLACEMENT_3D ( 'NONE', #12653, #113448, #92515 ) ;
#71706=ORIENTED_EDGE ( 'NONE', *, *, #88419, .T. ) ;
#71707=CARTESIAN_POINT ( 'NONE',  ( -3.950000000000028155, 12.50000000000000000, -6.776507416713039689 ) ) ;
#71708=CIRCLE ( 'NONE', #98893, 0.06509327318403745899 ) ;
#71709=ORIENTED_EDGE ( 'NONE', *, *, #31836, .F. ) ;
#71710=FACE_OUTER_BOUND ( 'NONE', #1628, .T. ) ;
#71711=ADVANCED_FACE ( 'NONE', ( #89968 ), #71625, .T. ) ;
#71712=CARTESIAN_POINT ( 'NONE',  ( 14.14999999999989200, 12.50000000000000000, -2.099970236277064473 ) ) ;
#71713=DIRECTION ( 'NONE',  ( 0.000000000000000000, 1.000000000000000000, 0.000000000000000000 ) ) ;
#71714=CARTESIAN_POINT ( 'NONE',  ( 3.149999999999946176, 2.500000000000000000, -6.841600689897077814 ) ) ;
#71715=DIRECTION ( 'NONE',  ( 0.000000000000000000, 0.000000000000000000, 1.000000000000000000 ) ) ;
#71716=CIRCLE ( 'NONE', #63303, 0.06509327318403745899 ) ;
#71717=ORIENTED_EDGE ( 'NONE', *, *, #53579, .T. ) ;
#71718=AXIS2_PLACEMENT_3D ( 'NONE', #58210, #59511, #98106 ) ;
#71719=CIRCLE ( 'NONE', #115618, 0.1000000000000002554 ) ;
#71720=EDGE_CURVE ( 'NONE', #127250, #71628, #35399, .T. ) ;
#71721=DIRECTION ( 'NONE',  ( -4.274815082592931898E-19, -0.9999939076577903929, -0.003490651415223739937 ) ) ;
#71722=CIRCLE ( 'NONE', #59223, 0.06509327318403745899 ) ;
#71723=DIRECTION ( 'NONE',  ( 0.000000000000000000, -0.000000000000000000, 1.000000000000000000 ) ) ;
#71724=VERTEX_POINT ( 'NONE', #121361 ) ;
#71725=VERTEX_POINT ( 'NONE', #110894 ) ;
#71726=ADVANCED_FACE ( 'NONE', ( #69692 ), #21901, .T. ) ;
#71727=EDGE_CURVE ( 'NONE', #32033, #51297, #77161, .T. ) ;
#71729=DIRECTION ( 'NONE',  ( 0.000000000000000000, 0.000000000000000000, 1.000000000000000000 ) ) ;
#71730=DIRECTION ( 'NONE',  ( -0.000000000000000000, -1.000000000000000000, -0.000000000000000000 ) ) ;
#71731=ADVANCED_FACE ( 'NONE', ( #52000 ), #101086, .T. ) ;
#71733=EDGE_CURVE ( 'NONE', #117143, #4956, #64635, .T. ) ;
#71734=VECTOR ( 'NONE', #93520, 1000.000000000000000 ) ;
#71735=DIRECTION ( 'NONE',  ( 0.000000000000000000, 1.000000000000000000, 0.000000000000000000 ) ) ;
#71736=DIRECTION ( 'NONE',  ( 0.000000000000000000, -0.000000000000000000, 1.000000000000000000 ) ) ;
#71737=CARTESIAN_POINT ( 'NONE',  ( -5.850000000000018296, 2.500000000000000000, 2.757883832488649656 ) ) ;
#71738=AXIS2_PLACEMENT_3D ( 'NONE', #117721, #20193, #40502 ) ;
#71739=DIRECTION ( 'NONE',  ( 0.000000000000000000, 1.000000000000000000, 0.000000000000000000 ) ) ;
#71740=CIRCLE ( 'NONE', #128084, 0.1000000000000002554 ) ;
#71741=AXIS2_PLACEMENT_3D ( 'NONE', #92118, #43064, #50279 ) ;
#71743=EDGE_CURVE ( 'NONE', #54236, #109083, #18664, .T. ) ;
#71744=EDGE_CURVE ( 'NONE', #92818, #16529, #39622, .T. ) ;
#71745=AXIS2_PLACEMENT_3D ( 'NONE', #122206, #93384, #102546 ) ;
#71746=EDGE_CURVE ( 'NONE', #39809, #19040, #98082, .T. ) ;
#71747=ADVANCED_FACE ( 'NONE', ( #51366 ), #85565, .T. ) ;
#71748=ADVANCED_FACE ( 'NONE', ( #120094 ), #30440, .T. ) ;
#71749=AXIS2_PLACEMENT_3D ( 'NONE', #65205, #105140, #34501 ) ;
#71750=VERTEX_POINT ( 'NONE', #20600 ) ;
#71751=CARTESIAN_POINT ( 'NONE',  ( 8.549999999999924327, 2.500000000000000000, 1.718653347947321386 ) ) ;
#71752=DIRECTION ( 'NONE',  ( -0.000000000000000000, -1.000000000000000000, -0.000000000000000000 ) ) ;
#71753=DIRECTION ( 'NONE',  ( 0.000000000000000000, 0.000000000000000000, 1.000000000000000000 ) ) ;
#71754=FACE_OUTER_BOUND ( 'NONE', #43905, .T. ) ;
#71755=ADVANCED_FACE ( 'NONE', ( #10742 ), #60547, .T. ) ;
#71756=VERTEX_POINT ( 'NONE', #2893 ) ;
#71757=CARTESIAN_POINT ( 'NONE',  ( 10.39999999999991154, 2.500000000000000000, -3.737306695894649700 ) ) ;
#71759=CARTESIAN_POINT ( 'NONE',  ( 3.099999999999944134, 2.500000000000000000, 4.676537180435972552 ) ) ;
#71760=EDGE_LOOP ( 'NONE', ( #43750, #62226, #9566, #23550 ) ) ;
#71761=VECTOR ( 'NONE', #23519, 1000.000000000000000 ) ;
#71762=ORIENTED_EDGE ( 'NONE', *, *, #8946, .F. ) ;
#71763=CARTESIAN_POINT ( 'NONE',  ( 14.59999999999989484, 2.500000000000000000, 0.6928203230275494784 ) ) ;
#71764=CIRCLE ( 'NONE', #11102, 0.1000000000000002554 ) ;
#71765=ORIENTED_EDGE ( 'NONE', *, *, #43687, .T. ) ;
#71766=CIRCLE ( 'NONE', #50836, 0.06509327318403745899 ) ;
#71767=ORIENTED_EDGE ( 'NONE', *, *, #48069, .F. ) ;
#71768=CARTESIAN_POINT ( 'NONE',  ( -1.650000000000035216, 2.500000000000000000, -1.372243186433550033 ) ) ;
#71769=AXIS2_PLACEMENT_3D ( 'NONE', #82964, #31298, #100644 ) ;
#71770=AXIS2_PLACEMENT_3D ( 'NONE', #64472, #124040, #15356 ) ;
#71771=LINE ( 'NONE', #41040, #101143 ) ;
#71772=CARTESIAN_POINT ( 'NONE',  ( -2.100000000000033396, 12.50000000000000000, -0.7579135962115917113 ) ) ;
#71773=CARTESIAN_POINT ( 'NONE',  ( -1.650000000000034772, 12.50000000000000000, 5.867463478539781896 ) ) ;
#71774=AXIS2_PLACEMENT_3D ( 'NONE', #3968, #116497, #66109 ) ;
#71776=CIRCLE ( 'NONE', #21594, 0.1000000000000002554 ) ;
#71777=AXIS2_PLACEMENT_3D ( 'NONE', #123311, #3540, #103686 ) ;
#71778=DIRECTION ( 'NONE',  ( -0.000000000000000000, -1.000000000000000000, -0.000000000000000000 ) ) ;
#71779=AXIS2_PLACEMENT_3D ( 'NONE', #106460, #114343, #75699 ) ;
#71780=EDGE_LOOP ( 'NONE', ( #41086, #81023, #94730, #101382 ) ) ;
#71781=AXIS2_PLACEMENT_3D ( 'NONE', #78658, #46598, #17775 ) ;
#71782=CARTESIAN_POINT ( 'NONE',  ( -4.350000000000023626, 2.500000000000000000, 2.511473670974873507 ) ) ;
#71783=CARTESIAN_POINT ( 'NONE',  ( 7.899999999999924860, 12.50000000000000000, 4.330127018922196314 ) ) ;
#71784=AXIS2_PLACEMENT_3D ( 'NONE', #121157, #129072, #21017 ) ;
#71785=ORIENTED_EDGE ( 'NONE', *, *, #44284, .F. ) ;
#71786=EDGE_CURVE ( 'NONE', #31778, #50468, #91836, .T. ) ;
#71787=EDGE_LOOP ( 'NONE', ( #48437, #63092 ) ) ;
#71788=ADVANCED_FACE ( 'NONE', ( #122660 ), #103012, .T. ) ;
#71789=ORIENTED_EDGE ( 'NONE', *, *, #86531, .T. ) ;
#71790=ORIENTED_EDGE ( 'NONE', *, *, #58101, .T. ) ;
#71791=DIRECTION ( 'NONE',  ( 0.000000000000000000, 0.000000000000000000, -1.000000000000000000 ) ) ;
#71792=FACE_OUTER_BOUND ( 'NONE', #34496, .T. ) ;
#71793=PLANE ( 'NONE',  #54628 ) ;
#71794=FACE_BOUND ( 'NONE', #119716, .T. ) ;
#71795=ORIENTED_EDGE ( 'NONE', *, *, #4311, .T. ) ;
#71796=LINE ( 'NONE', #5444, #80876 ) ;
#71798=DIRECTION ( 'NONE',  ( 0.000000000000000000, 0.000000000000000000, 1.000000000000000000 ) ) ;
#71799=CARTESIAN_POINT ( 'NONE',  ( 7.949999999999925571, 2.500000000000000000, -6.395190528383301931 ) ) ;
#71800=AXIS2_PLACEMENT_3D ( 'NONE', #57120, #28318, #126519 ) ;
#71801=ADVANCED_FACE ( 'NONE', ( #42847 ), #25100, .T. ) ;
#71802=LINE ( 'NONE', #60699, #111259 ) ;
#71804=LINE ( 'NONE', #103188, #49209 ) ;
#71805=CONICAL_SURFACE ( 'NONE', #94783, 0.09999999999999982514, 0.003490658503988666988 ) ;
#71806=AXIS2_PLACEMENT_3D ( 'NONE', #23970, #26546, #4951 ) ;
#71807=DIRECTION ( 'NONE',  ( -0.000000000000000000, -1.000000000000000000, -0.000000000000000000 ) ) ;
#71808=ORIENTED_EDGE ( 'NONE', *, *, #28275, .T. ) ;
#71809=VERTEX_POINT ( 'NONE', #74210 ) ;
#71810=VERTEX_POINT ( 'NONE', #43473 ) ;
#71811=EDGE_LOOP ( 'NONE', ( #102106, #126898, #68910, #45099 ) ) ;
#71812=VERTEX_POINT ( 'NONE', #114130 ) ;
#71813=CARTESIAN_POINT ( 'NONE',  ( 3.949999999999941558, 2.500000000000000000, -1.718653347947326049 ) ) ;
#71814=CARTESIAN_POINT ( 'NONE',  ( -3.750000000000027534, 2.500000000000000000, 2.857883832488649301 ) ) ;
#71815=ORIENTED_EDGE ( 'NONE', *, *, #49541, .T. ) ;
#71816=FACE_BOUND ( 'NONE', #25798, .T. ) ;
#71817=VECTOR ( 'NONE', #11077, 1000.000000000000000 ) ;
#71818=AXIS2_PLACEMENT_3D ( 'NONE', #66551, #75101, #106490 ) ;
#71819=FACE_OUTER_BOUND ( 'NONE', #117384, .T. ) ;
#71820=AXIS2_PLACEMENT_3D ( 'NONE', #35155, #75061, #16109 ) ;
#71821=AXIS2_PLACEMENT_3D ( 'NONE', #94281, #52430, #81257 ) ;
#71822=ORIENTED_EDGE ( 'NONE', *, *, #27956, .T. ) ;
#71824=CARTESIAN_POINT ( 'NONE',  ( 2.899999999999946620, 2.500000000000000000, -5.122947341949753763 ) ) ;
#71825=CARTESIAN_POINT ( 'NONE',  ( 9.349999999999916156, 12.50000000000000000, 6.841600689897072485 ) ) ;
#71826=DIRECTION ( 'NONE',  ( 0.000000000000000000, 1.000000000000000000, 0.000000000000000000 ) ) ;
#71827=CONICAL_SURFACE ( 'NONE', #15363, 0.1000000000000002554, 0.003490658503988666988 ) ;
#71828=ORIENTED_EDGE ( 'NONE', *, *, #38032, .T. ) ;
#71829=CARTESIAN_POINT ( 'NONE',  ( -5.850000000000022737, 12.50000000000000000, -2.165063509461101710 ) ) ;
#71830=EDGE_CURVE ( 'NONE', #97166, #84391, #29150, .T. ) ;
#71831=ORIENTED_EDGE ( 'NONE', *, *, #30894, .F. ) ;
#71832=AXIS2_PLACEMENT_3D ( 'NONE', #28503, #109640, #11428 ) ;
#71833=VECTOR ( 'NONE', #48717, 1000.000000000000000 ) ;
#71834=ORIENTED_EDGE ( 'NONE', *, *, #126281, .T. ) ;
#71835=ORIENTED_EDGE ( 'NONE', *, *, #119046, .T. ) ;
#71836=CARTESIAN_POINT ( 'NONE',  ( -5.600000000000023626, 2.500000000000000000, -4.083716857408426826 ) ) ;
#71837=DIRECTION ( 'NONE',  ( 0.000000000000000000, 1.000000000000000000, 0.000000000000000000 ) ) ;
#71838=CONICAL_SURFACE ( 'NONE', #99018, 0.1000000000000002554, 0.003490658503988666988 ) ;
#71839=ORIENTED_EDGE ( 'NONE', *, *, #128749, .T. ) ;
#71840=CARTESIAN_POINT ( 'NONE',  ( 0.1999999999999562961, 2.500000000000000000, 4.676537180435972552 ) ) ;
#71841=VECTOR ( 'NONE', #32387, 1000.000000000000000 ) ;
#71842=DIRECTION ( 'NONE',  ( 0.000000000000000000, 1.000000000000000000, 0.000000000000000000 ) ) ;
#71843=DIRECTION ( 'NONE',  ( -0.000000000000000000, 1.000000000000000000, -0.000000000000000000 ) ) ;
#71844=DIRECTION ( 'NONE',  ( -0.000000000000000000, -1.000000000000000000, -0.000000000000000000 ) ) ;
#71846=VERTEX_POINT ( 'NONE', #94475 ) ;
#71847=EDGE_CURVE ( 'NONE', #93896, #78285, #3983, .T. ) ;
#71848=DIRECTION ( 'NONE',  ( 0.000000000000000000, 1.000000000000000000, 0.000000000000000000 ) ) ;
#71849=EDGE_CURVE ( 'NONE', #39661, #74932, #5451, .T. ) ;
#71850=ORIENTED_EDGE ( 'NONE', *, *, #109904, .T. ) ;
#71852=VERTEX_POINT ( 'NONE', #53924 ) ;
#71853=DIRECTION ( 'NONE',  ( -0.000000000000000000, 1.000000000000000000, -0.000000000000000000 ) ) ;
#71854=ORIENTED_EDGE ( 'NONE', *, *, #61346, .F. ) ;
#71855=CARTESIAN_POINT ( 'NONE',  ( -6.050000000000022027, 2.500000000000000000, -6.148780366869526226 ) ) ;
#71856=DIRECTION ( 'NONE',  ( 0.000000000000000000, 1.000000000000000000, 0.000000000000000000 ) ) ;
#71857=CARTESIAN_POINT ( 'NONE',  ( -7.100000000000018296, 12.50000000000000000, -2.385244779468109755E-15 ) ) ;
#71858=AXIS2_PLACEMENT_3D ( 'NONE', #91619, #13037, #22261 ) ;
#71859=DIRECTION ( 'NONE',  ( 0.000000000000000000, -0.000000000000000000, 1.000000000000000000 ) ) ;
#71860=EDGE_CURVE ( 'NONE', #120640, #125450, #110602, .T. ) ;
#71861=FACE_OUTER_BOUND ( 'NONE', #26858, .T. ) ;
#71862=ORIENTED_EDGE ( 'NONE', *, *, #81342, .F. ) ;
#71863=EDGE_LOOP ( 'NONE', ( #47127, #22449, #65717, #71515 ) ) ;
#71864=CARTESIAN_POINT ( 'NONE',  ( -8.100000000000013856, 2.500000000000000000, 0.3464101615137736845 ) ) ;
#71865=AXIS2_PLACEMENT_3D ( 'NONE', #12034, #91250, #91896 ) ;
#71866=CONICAL_SURFACE ( 'NONE', #103149, 0.09999999999999982514, 0.003490658503988666988 ) ;
#71867=AXIS2_PLACEMENT_3D ( 'NONE', #121544, #1138, #60081 ) ;
#71868=DIRECTION ( 'NONE',  ( 0.000000000000000000, -0.9999939076577903929, 0.003490651415223739937 ) ) ;
#71869=CIRCLE ( 'NONE', #46729, 0.06509327318403745899 ) ;
#71870=VECTOR ( 'NONE', #3472, 1000.000000000000000 ) ;
#71871=CARTESIAN_POINT ( 'NONE',  ( 0.5999999999999621192, 12.50000000000000000, 0.3464101615137758494 ) ) ;
#71872=EDGE_LOOP ( 'NONE', ( #55777, #60570 ) ) ;
#71873=ORIENTED_EDGE ( 'NONE', *, *, #52156, .F. ) ;
#71874=EDGE_LOOP ( 'NONE', ( #2610, #23224 ) ) ;
#71875=CARTESIAN_POINT ( 'NONE',  ( -4.600000000000024514, 12.50000000000000000, -0.6928203230275542523 ) ) ;
#71876=ORIENTED_EDGE ( 'NONE', *, *, #103124, .F. ) ;
#71877=CARTESIAN_POINT ( 'NONE',  ( 8.749999999999920064, 2.500000000000000000, -2.857883832488653741 ) ) ;
#71878=PLANE ( 'NONE',  #116670 ) ;
#71879=CIRCLE ( 'NONE', #103266, 0.06509327318403745899 ) ;
#71880=CONICAL_SURFACE ( 'NONE', #76075, 0.1000000000000000472, 0.003490658503988666988 ) ;
#71881=FACE_OUTER_BOUND ( 'NONE', #23347, .T. ) ;
#71882=CARTESIAN_POINT ( 'NONE',  ( -6.050000000000022027, 2.500000000000000000, -1.818653347947326138 ) ) ;
#71883=LINE ( 'NONE', #50956, #59132 ) ;
#71884=DIRECTION ( 'NONE',  ( 0.000000000000000000, 1.000000000000000000, 0.000000000000000000 ) ) ;
#71885=CARTESIAN_POINT ( 'NONE',  ( 9.599999999999917932, 12.50000000000000000, 0.7579135962115869374 ) ) ;
#71886=VECTOR ( 'NONE', #30849, 1000.000000000000000 ) ;
#71887=DIRECTION ( 'NONE',  ( 0.000000000000000000, 0.000000000000000000, 1.000000000000000000 ) ) ;
#71888=VERTEX_POINT ( 'NONE', #33012 ) ;
#71889=EDGE_CURVE ( 'NONE', #34976, #4024, #15914, .T. ) ;
#71890=CARTESIAN_POINT ( 'NONE',  ( -9.350000000000006750, 2.500000000000000000, 1.818653347947321475 ) ) ;
#71891=CARTESIAN_POINT ( 'NONE',  ( 59.88087687668669901, -3.776023963385989557, 4.996435080087643144 ) ) ;
#71892=ORIENTED_EDGE ( 'NONE', *, *, #25025, .T. ) ;
#71893=ORIENTED_EDGE ( 'NONE', *, *, #43491, .T. ) ;
#71894=ADVANCED_FACE ( 'NONE', ( #4152 ), #22886, .T. ) ;
#71896=PLANE ( 'NONE',  #76162 ) ;
#71897=CARTESIAN_POINT ( 'NONE',  ( 7.099999999999925926, 2.500000000000000000, 0.7928203230275495672 ) ) ;
#71898=EDGE_CURVE ( 'NONE', #62131, #25372, #65005, .T. ) ;
#71899=CIRCLE ( 'NONE', #50973, 0.06509327318403745899 ) ;
#71900=DIRECTION ( 'NONE',  ( -0.000000000000000000, -1.000000000000000000, -0.000000000000000000 ) ) ;
#71901=CARTESIAN_POINT ( 'NONE',  ( -6.250000000000015987, 2.500000000000000000, 1.372243186433545370 ) ) ;
#71902=CARTESIAN_POINT ( 'NONE',  ( 15.19999999999989271, 2.500000000000000000, -0.2464101615137783419 ) ) ;
#71903=DIRECTION ( 'NONE',  ( 0.000000000000000000, 0.000000000000000000, 1.000000000000000000 ) ) ;
#71904=FACE_OUTER_BOUND ( 'NONE', #123428, .T. ) ;
#71905=EDGE_CURVE ( 'NONE', #123378, #26594, #93894, .T. ) ;
#71906=EDGE_CURVE ( 'NONE', #41184, #34349, #70909, .T. ) ;
#71907=EDGE_CURVE ( 'NONE', #109647, #30034, #25744, .T. ) ;
#71908=CIRCLE ( 'NONE', #17489, 0.09999999999999982514 ) ;
#71909=CARTESIAN_POINT ( 'NONE',  ( 8.949999999999921130, 12.50000000000000000, 1.818653347947321475 ) ) ;
#71910=AXIS2_PLACEMENT_3D ( 'NONE', #120587, #62324, #110754 ) ;
#71911=ORIENTED_EDGE ( 'NONE', *, *, #46574, .F. ) ;
#71912=CONICAL_SURFACE ( 'NONE', #111604, 0.09999999999999999167, 0.003490658503988666988 ) ;
#71913=VERTEX_POINT ( 'NONE', #84014 ) ;
#71914=EDGE_CURVE ( 'NONE', #66570, #120306, #63094, .T. ) ;
#71915=ORIENTED_EDGE ( 'NONE', *, *, #41419, .F. ) ;
#71916=ORIENTED_EDGE ( 'NONE', *, *, #28106, .T. ) ;
#71917=VECTOR ( 'NONE', #116859, 1000.000000000000000 ) ;
#71918=DIRECTION ( 'NONE',  ( 0.000000000000000000, 1.000000000000000000, 0.000000000000000000 ) ) ;
#71919=DIRECTION ( 'NONE',  ( -0.000000000000000000, -1.000000000000000000, -0.000000000000000000 ) ) ;
#71920=ADVANCED_FACE ( 'NONE', ( #33643 ), #23823, .T. ) ;
#71921=VECTOR ( 'NONE', #14033, 1000.000000000000000 ) ;
#71922=ORIENTED_EDGE ( 'NONE', *, *, #45751, .T. ) ;
#71923=CARTESIAN_POINT ( 'NONE',  ( 14.14999999999989555, 12.50000000000000000, 2.165063509461097713 ) ) ;
#71924=AXIS2_PLACEMENT_3D ( 'NONE', #92036, #120219, #110386 ) ;
#71925=CARTESIAN_POINT ( 'NONE',  ( 5.849999999999932143, 2.500000000000000000, 1.472243186433545459 ) ) ;
#71926=DIRECTION ( 'NONE',  ( 0.000000000000000000, 1.000000000000000000, 0.000000000000000000 ) ) ;
#71927=EDGE_LOOP ( 'NONE', ( #5365, #108833 ) ) ;
#71928=LINE ( 'NONE', #111845, #47452 ) ;
#71929=DIRECTION ( 'NONE',  ( -0.000000000000000000, 1.000000000000000000, -0.000000000000000000 ) ) ;
#71930=ORIENTED_EDGE ( 'NONE', *, *, #121424, .F. ) ;
#71931=CONICAL_SURFACE ( 'NONE', #84437, 0.1000000000000002554, 0.003490658503988666988 ) ;
#71932=AXIS2_PLACEMENT_3D ( 'NONE', #107526, #17849, #28329 ) ;
#71933=ORIENTED_EDGE ( 'NONE', *, *, #6090, .F. ) ;
#71934=EDGE_LOOP ( 'NONE', ( #5507, #67775, #94574, #60460 ) ) ;
#71935=ORIENTED_EDGE ( 'NONE', *, *, #97659, .F. ) ;
#71936=DIRECTION ( 'NONE',  ( -0.000000000000000000, 1.000000000000000000, -0.000000000000000000 ) ) ;
#71937=CONICAL_SURFACE ( 'NONE', #113693, 0.09999999999999982514, 0.003490658503988666988 ) ;
#71938=CARTESIAN_POINT ( 'NONE',  ( -8.950000000000009948, 2.500000000000000000, -6.741600689897071952 ) ) ;
#71939=CARTESIAN_POINT ( 'NONE',  ( 2.500000000000002220, -1.500000000000000000, -9.999999999999998224 ) ) ;
#71940=AXIS2_PLACEMENT_3D ( 'NONE', #28659, #118311, #118955 ) ;
#71941=EDGE_LOOP ( 'NONE', ( #54098, #5929 ) ) ;
#71942=CARTESIAN_POINT ( 'NONE',  ( 12.89999999999990266, 2.500000000000000000, -3.737306695894649700 ) ) ;
#71943=ORIENTED_EDGE ( 'NONE', *, *, #104727, .T. ) ;
#71944=DIRECTION ( 'NONE',  ( -0.000000000000000000, 1.000000000000000000, -0.000000000000000000 ) ) ;
#71945=DIRECTION ( 'NONE',  ( 0.000000000000000000, 1.000000000000000000, 0.000000000000000000 ) ) ;
#71946=DIRECTION ( 'NONE',  ( 0.000000000000000000, -0.9999939076577903929, 0.003490651415223739937 ) ) ;
#71947=FACE_OUTER_BOUND ( 'NONE', #98240, .T. ) ;
#71948=ORIENTED_EDGE ( 'NONE', *, *, #45210, .T. ) ;
#71949=EDGE_CURVE ( 'NONE', #18148, #29100, #45867, .T. ) ;
#71950=VERTEX_POINT ( 'NONE', #26410 ) ;
#71951=VERTEX_POINT ( 'NONE', #46047 ) ;
#71952=LINE ( 'NONE', #128463, #20999 ) ;
#71953=DIRECTION ( 'NONE',  ( 0.000000000000000000, 0.000000000000000000, 1.000000000000000000 ) ) ;
#71954=CIRCLE ( 'NONE', #61586, 0.06509327318403741736 ) ;
#71955=AXIS2_PLACEMENT_3D ( 'NONE', #7090, #57506, #28694 ) ;
#71956=CARTESIAN_POINT ( 'NONE',  ( -0.8500000000000382805, 2.500000000000000000, -1.572243186433550211 ) ) ;
#71957=FACE_BOUND ( 'NONE', #45231, .T. ) ;
#71958=CARTESIAN_POINT ( 'NONE',  ( -0.6000000000000323963, 2.500000000000000000, 0.3464101615137759604 ) ) ;
#71959=CARTESIAN_POINT ( 'NONE',  ( -10.84999999999999964, 12.50000000000000000, 1.472243186433545459 ) ) ;
#71960=CARTESIAN_POINT ( 'NONE',  ( -15.79999999999998117, 2.500000000000000000, 0.000000000000000000 ) ) ;
#71961=ADVANCED_FACE ( 'NONE', ( #7382 ), #19125, .T. ) ;
#71962=AXIS2_PLACEMENT_3D ( 'NONE', #48597, #95762, #27636 ) ;
#71963=AXIS2_PLACEMENT_3D ( 'NONE', #68503, #8926, #85571 ) ;
#71964=CIRCLE ( 'NONE', #13349, 0.09999999999999982514 ) ;
#71965=AXIS2_PLACEMENT_3D ( 'NONE', #58659, #8889, #18069 ) ;
#71966=DIRECTION ( 'NONE',  ( 0.000000000000000000, 1.000000000000000000, 0.000000000000000000 ) ) ;
#71968=DIRECTION ( 'NONE',  ( 0.000000000000000000, 0.000000000000000000, -1.000000000000000000 ) ) ;
#71969=ORIENTED_EDGE ( 'NONE', *, *, #35434, .F. ) ;
#71970=CIRCLE ( 'NONE', #115861, 0.06509327318403745899 ) ;
#71971=DIRECTION ( 'NONE',  ( -0.000000000000000000, -1.000000000000000000, -0.000000000000000000 ) ) ;
#71972=CIRCLE ( 'NONE', #103360, 2.000000000000000000 ) ;
#71973=FACE_OUTER_BOUND ( 'NONE', #111948, .T. ) ;
#71974=ORIENTED_EDGE ( 'NONE', *, *, #87411, .T. ) ;
#71975=ORIENTED_EDGE ( 'NONE', *, *, #8617, .F. ) ;
#71976=CIRCLE ( 'NONE', #32283, 0.09999999999999982514 ) ;
#71977=PLANE ( 'NONE',  #31403 ) ;
#71978=FACE_OUTER_BOUND ( 'NONE', #20775, .T. ) ;
#71979=FACE_BOUND ( 'NONE', #12983, .T. ) ;
#71980=LINE ( 'NONE', #81770, #38940 ) ;
#71981=EDGE_LOOP ( 'NONE', ( #72004, #45292, #114030, #3271 ) ) ;
#71982=CARTESIAN_POINT ( 'NONE',  ( 12.09999999999990550, 12.50000000000000000, -3.637306695894650055 ) ) ;
#71983=DIRECTION ( 'NONE',  ( 0.000000000000000000, 0.000000000000000000, 1.000000000000000000 ) ) ;
#71984=CIRCLE ( 'NONE', #15524, 0.09999999999999982514 ) ;
#71985=ORIENTED_EDGE ( 'NONE', *, *, #89935, .F. ) ;
#71986=FACE_OUTER_BOUND ( 'NONE', #98202, .T. ) ;
#71987=PLANE ( 'NONE',  #72101 ) ;
#71988=EDGE_CURVE ( 'NONE', #111575, #117378, #33271, .T. ) ;
#71989=ORIENTED_EDGE ( 'NONE', *, *, #128331, .F. ) ;
#71990=DIRECTION ( 'NONE',  ( -0.000000000000000000, 1.000000000000000000, -0.000000000000000000 ) ) ;
#71991=CARTESIAN_POINT ( 'NONE',  ( -3.950000000000026379, 2.500000000000000000, 6.941600689897073018 ) ) ;
#71992=CIRCLE ( 'NONE', #120016, 0.1000000000000002554 ) ;
#71993=EDGE_CURVE ( 'NONE', #95287, #70361, #127812, .T. ) ;
#71994=AXIS2_PLACEMENT_3D ( 'NONE', #92898, #73885, #4468 ) ;
#71995=ORIENTED_EDGE ( 'NONE', *, *, #105840, .T. ) ;
#71996=CARTESIAN_POINT ( 'NONE',  ( -3.950000000000026379, 12.50000000000000000, -1.818653347947326138 ) ) ;
#71997=CARTESIAN_POINT ( 'NONE',  ( -8.150000000000012790, 2.500000000000000000, -2.411473670974877859 ) ) ;
#71998=DIRECTION ( 'NONE',  ( 0.000000000000000000, 0.000000000000000000, -1.000000000000000000 ) ) ;
#71999=EDGE_LOOP ( 'NONE', ( #39208, #28220 ) ) ;
#72000=ADVANCED_FACE ( 'NONE', ( #47983 ), #57798, .T. ) ;
#72001=VERTEX_POINT ( 'NONE', #6089 ) ;
#72002=EDGE_CURVE ( 'NONE', #17444, #120069, #123132, .T. ) ;
#72003=DIRECTION ( 'NONE',  ( 0.000000000000000000, 0.000000000000000000, -1.000000000000000000 ) ) ;
#72004=ORIENTED_EDGE ( 'NONE', *, *, #45111, .F. ) ;
#72005=FACE_OUTER_BOUND ( 'NONE', #5748, .T. ) ;
#72006=CARTESIAN_POINT ( 'NONE',  ( -8.950000000000009948, 12.50000000000000000, -1.818653347947326138 ) ) ;
#72007=VECTOR ( 'NONE', #46158, 1000.000000000000000 ) ;
#72008=LINE ( 'NONE', #61545, #80134 ) ;
#72009=EDGE_LOOP ( 'NONE', ( #52369, #14817 ) ) ;
#72010=ADVANCED_FACE ( 'NONE', ( #108165 ), #43738, .T. ) ;
#72011=CARTESIAN_POINT ( 'NONE',  ( -13.09999999999999254, 2.500000000000000000, -4.676537180435975216 ) ) ;
#72012=FACE_OUTER_BOUND ( 'NONE', #82381, .T. ) ;
#72013=CARTESIAN_POINT ( 'NONE',  ( 8.349999999999919709, 12.50000000000000000, -2.857883832488653741 ) ) ;
#72014=DIRECTION ( 'NONE',  ( -0.000000000000000000, -1.000000000000000000, -0.000000000000000000 ) ) ;
#72015=FACE_OUTER_BOUND ( 'NONE', #91205, .T. ) ;
#72016=EDGE_CURVE ( 'NONE', #109879, #113918, #100153, .T. ) ;
#72017=DIRECTION ( 'NONE',  ( 0.000000000000000000, 0.000000000000000000, 1.000000000000000000 ) ) ;
#72018=VERTEX_POINT ( 'NONE', #8659 ) ;
#72019=ORIENTED_EDGE ( 'NONE', *, *, #91207, .F. ) ;
#72020=CARTESIAN_POINT ( 'NONE',  ( 11.64999999999990443, 2.500000000000000000, 1.572243186433545548 ) ) ;
#72021=CIRCLE ( 'NONE', #88730, 0.06509327318403745899 ) ;
#72022=EDGE_LOOP ( 'NONE', ( #88007, #66116 ) ) ;
#72023=CIRCLE ( 'NONE', #3062, 0.1000000000000002554 ) ;
#72025=VERTEX_POINT ( 'NONE', #86591 ) ;
#72026=VERTEX_POINT ( 'NONE', #48617 ) ;
#72027=VERTEX_POINT ( 'NONE', #107535 ) ;
#72028=CIRCLE ( 'NONE', #42801, 0.06509327318403745899 ) ;
#72029=CARTESIAN_POINT ( 'NONE',  ( 2.049999999999948308, 2.500000000000000000, 6.495190528383297135 ) ) ;
#72030=AXIS2_PLACEMENT_3D ( 'NONE', #49436, #108328, #89345 ) ;
#72031=CARTESIAN_POINT ( 'NONE',  ( 1.899999999999949507, 2.500000000000000000, 4.776537180435972196 ) ) ;
#72032=DIRECTION ( 'NONE',  ( 0.000000000000000000, -0.000000000000000000, 1.000000000000000000 ) ) ;
#72033=FACE_OUTER_BOUND ( 'NONE', #116882, .T. ) ;
#72034=LINE ( 'NONE', #9881, #85635 ) ;
#72035=CARTESIAN_POINT ( 'NONE',  ( -1.250000000000001554, 2.500000000000000000, 2.065063509461097624 ) ) ;
#72036=DIRECTION ( 'NONE',  ( 0.000000000000000000, 1.000000000000000000, 0.000000000000000000 ) ) ;
#72037=DIRECTION ( 'NONE',  ( -0.000000000000000000, 1.000000000000000000, -0.000000000000000000 ) ) ;
#72038=FACE_OUTER_BOUND ( 'NONE', #5766, .T. ) ;
#72039=EDGE_LOOP ( 'NONE', ( #57208, #306 ) ) ;
#72040=EDGE_CURVE ( 'NONE', #11303, #125704, #37468, .T. ) ;
#72041=AXIS2_PLACEMENT_3D ( 'NONE', #76707, #57050, #26329 ) ;
#72042=AXIS2_PLACEMENT_3D ( 'NONE', #38425, #78345, #18756 ) ;
#72043=DIRECTION ( 'NONE',  ( 0.000000000000000000, -0.000000000000000000, 1.000000000000000000 ) ) ;
#72044=AXIS2_PLACEMENT_3D ( 'NONE', #46233, #58005, #127384 ) ;
#72045=ORIENTED_EDGE ( 'NONE', *, *, #64059, .F. ) ;
#72046=ORIENTED_EDGE ( 'NONE', *, *, #10720, .F. ) ;
#72047=DIRECTION ( 'NONE',  ( 0.000000000000000000, 0.000000000000000000, 1.000000000000000000 ) ) ;
#72048=DIRECTION ( 'NONE',  ( 0.000000000000000000, 1.000000000000000000, 0.000000000000000000 ) ) ;
#72049=PLANE ( 'NONE',  #34026 ) ;
#72050=EDGE_CURVE ( 'NONE', #74488, #73563, #87612, .T. ) ;
#72051=AXIS2_PLACEMENT_3D ( 'NONE', #120327, #39855, #30676 ) ;
#72052=DIRECTION ( 'NONE',  ( 0.000000000000000000, -0.000000000000000000, 1.000000000000000000 ) ) ;
#72053=CIRCLE ( 'NONE', #72343, 0.1000000000000002554 ) ;
#72054=CIRCLE ( 'NONE', #124278, 0.1000000000000000056 ) ;
#72055=DIRECTION ( 'NONE',  ( 0.000000000000000000, 1.000000000000000000, 0.000000000000000000 ) ) ;
#72056=CARTESIAN_POINT ( 'NONE',  ( 4.599999999999939249, 2.500000000000000000, -3.637306695894650055 ) ) ;
#72057=DIRECTION ( 'NONE',  ( -0.000000000000000000, -1.000000000000000000, -0.000000000000000000 ) ) ;
#72058=ORIENTED_EDGE ( 'NONE', *, *, #121799, .F. ) ;
#72059=EDGE_CURVE ( 'NONE', #109722, #73210, #48021, .T. ) ;
#72060=AXIS2_PLACEMENT_3D ( 'NONE', #58239, #86383, #118424 ) ;
#72061=EDGE_CURVE ( 'NONE', #29100, #73228, #28986, .T. ) ;
#72062=EDGE_CURVE ( 'NONE', #77164, #122473, #114888, .T. ) ;
#72063=CIRCLE ( 'NONE', #113916, 0.1000000000000000472 ) ;
#72064=ORIENTED_EDGE ( 'NONE', *, *, #40132, .T. ) ;
#72065=CIRCLE ( 'NONE', #53284, 0.06509327318403745899 ) ;
#72066=VERTEX_POINT ( 'NONE', #66312 ) ;
#72067=ADVANCED_FACE ( 'NONE', ( #106245 ), #127437, .T. ) ;
#72068=EDGE_LOOP ( 'NONE', ( #38131, #99986 ) ) ;
#72069=VECTOR ( 'NONE', #38431, 1000.000000000000000 ) ;
#72070=ORIENTED_EDGE ( 'NONE', *, *, #9898, .F. ) ;
#72072=DIRECTION ( 'NONE',  ( 0.000000000000000000, 1.000000000000000000, 0.000000000000000000 ) ) ;
#72073=EDGE_CURVE ( 'NONE', #54151, #19741, #70993, .T. ) ;
#72074=EDGE_CURVE ( 'NONE', #57754, #12097, #121165, .T. ) ;
#72075=CARTESIAN_POINT ( 'NONE',  ( -5.650000000000023448, 2.500000000000000000, -1.818653347947326138 ) ) ;
#72076=DIRECTION ( 'NONE',  ( 0.000000000000000000, 0.000000000000000000, 1.000000000000000000 ) ) ;
#72077=FACE_OUTER_BOUND ( 'NONE', #81688, .T. ) ;
#72078=VERTEX_POINT ( 'NONE', #17183 ) ;
#72079=CARTESIAN_POINT ( 'NONE',  ( 4.799999999999935874, 2.500000000000000000, 0.3464101615137735735 ) ) ;
#72080=FACE_OUTER_BOUND ( 'NONE', #8858, .T. ) ;
#72081=CARTESIAN_POINT ( 'NONE',  ( -6.900000000000015454, 12.50000000000000000, 4.676537180435972552 ) ) ;
#72082=CARTESIAN_POINT ( 'NONE',  ( 0.4499999999999569344, 12.50000000000000000, -2.165063509461101710 ) ) ;
#72083=VECTOR ( 'NONE', #94413, 1000.000000000000000 ) ;
#72084=DIRECTION ( 'NONE',  ( 0.000000000000000000, 0.000000000000000000, 1.000000000000000000 ) ) ;
#72085=ORIENTED_EDGE ( 'NONE', *, *, #27937, .T. ) ;
#72086=ORIENTED_EDGE ( 'NONE', *, *, #80627, .F. ) ;
#72087=ORIENTED_EDGE ( 'NONE', *, *, #20456, .F. ) ;
#72088=CARTESIAN_POINT ( 'NONE',  ( 6.449999999999931788, 2.500000000000000000, -2.511473670974877948 ) ) ;
#72089=VERTEX_POINT ( 'NONE', #57141 ) ;
#72090=CONICAL_SURFACE ( 'NONE', #69932, 0.09999999999999999167, 0.003490658503988666988 ) ;
#72091=DIRECTION ( 'NONE',  ( 0.000000000000000000, 0.000000000000000000, 1.000000000000000000 ) ) ;
#72092=DIRECTION ( 'NONE',  ( -0.000000000000000000, -1.000000000000000000, -0.000000000000000000 ) ) ;
#72093=AXIS2_PLACEMENT_3D ( 'NONE', #89504, #68566, #119596 ) ;
#72094=ORIENTED_EDGE ( 'NONE', *, *, #101275, .F. ) ;
#72095=CARTESIAN_POINT ( 'NONE',  ( 7.299999999999926104, 2.500000000000000000, -0.2464101615137782308 ) ) ;
#72096=DIRECTION ( 'NONE',  ( 0.000000000000000000, 0.000000000000000000, -1.000000000000000000 ) ) ;
#72097=DIRECTION ( 'NONE',  ( -0.000000000000000000, -1.000000000000000000, -0.000000000000000000 ) ) ;
#72098=DIRECTION ( 'NONE',  ( -4.274815082592931898E-19, -0.9999939076577903929, -0.003490651415223739937 ) ) ;
#72099=CONICAL_SURFACE ( 'NONE', #57427, 0.1000000000000002554, 0.003490658503988666988 ) ;
#72100=DIRECTION ( 'NONE',  ( 0.000000000000000000, 0.000000000000000000, 1.000000000000000000 ) ) ;
#72101=AXIS2_PLACEMENT_3D ( 'NONE', #2562, #90304, #80521 ) ;
#72102=ORIENTED_EDGE ( 'NONE', *, *, #110520, .F. ) ;
#72103=VERTEX_POINT ( 'NONE', #97066 ) ;
#72105=DIRECTION ( 'NONE',  ( 0.000000000000000000, 0.000000000000000000, -1.000000000000000000 ) ) ;
#72106=DIRECTION ( 'NONE',  ( -0.000000000000000000, 1.000000000000000000, -0.000000000000000000 ) ) ;
#72107=FACE_OUTER_BOUND ( 'NONE', #37668, .T. ) ;
#72108=ADVANCED_FACE ( 'NONE', ( #127191 ), #32219, .T. ) ;
#72109=ORIENTED_EDGE ( 'NONE', *, *, #47643, .F. ) ;
#72110=AXIS2_PLACEMENT_3D ( 'NONE', #101772, #12090, #91948 ) ;
#72111=EDGE_LOOP ( 'NONE', ( #17237, #3447, #59749, #97898 ) ) ;
#72112=DIRECTION ( 'NONE',  ( 0.000000000000000000, 1.000000000000000000, 0.000000000000000000 ) ) ;
#72113=CARTESIAN_POINT ( 'NONE',  ( 13.09999999999989839, 2.500000000000000000, -0.2464101615137783419 ) ) ;
#72114=DIRECTION ( 'NONE',  ( 0.000000000000000000, 0.000000000000000000, 1.000000000000000000 ) ) ;
#72115=AXIS2_PLACEMENT_3D ( 'NONE', #12689, #2229, #80166 ) ;
#72116=DIRECTION ( 'NONE',  ( -0.000000000000000000, 1.000000000000000000, -0.000000000000000000 ) ) ;
#72117=ORIENTED_EDGE ( 'NONE', *, *, #17098, .T. ) ;
#72118=DIRECTION ( 'NONE',  ( -0.000000000000000000, 1.000000000000000000, -0.000000000000000000 ) ) ;
#72119=FACE_OUTER_BOUND ( 'NONE', #77092, .T. ) ;
#72120=ORIENTED_EDGE ( 'NONE', *, *, #97039, .T. ) ;
#72121=CARTESIAN_POINT ( 'NONE',  ( -8.150000000000014566, 2.500000000000000000, -6.741600689897072840 ) ) ;
#72122=ORIENTED_EDGE ( 'NONE', *, *, #34704, .F. ) ;
#72123=DIRECTION ( 'NONE',  ( 0.000000000000000000, 0.000000000000000000, 1.000000000000000000 ) ) ;
#72124=AXIS2_PLACEMENT_3D ( 'NONE', #85715, #96178, #68016 ) ;
#72125=ORIENTED_EDGE ( 'NONE', *, *, #56952, .T. ) ;
#72126=CARTESIAN_POINT ( 'NONE',  ( 11.64999999999990621, 2.500000000000000000, 6.395190528383296602 ) ) ;
#72128=CIRCLE ( 'NONE', #30376, 0.06509327318403745899 ) ;
#72129=CIRCLE ( 'NONE', #17827, 0.06509327318403745899 ) ;
#72131=ORIENTED_EDGE ( 'NONE', *, *, #73614, .F. ) ;
#72132=DIRECTION ( 'NONE',  ( 0.000000000000000000, 0.000000000000000000, 1.000000000000000000 ) ) ;
#72133=DIRECTION ( 'NONE',  ( 0.000000000000000000, 0.000000000000000000, -1.000000000000000000 ) ) ;
#72134=CARTESIAN_POINT ( 'NONE',  ( -6.517459502904499961E-15, 2.500000000000000000, 4.230127018922196669 ) ) ;
#72136=VECTOR ( 'NONE', #61541, 1000.000000000000000 ) ;
#72137=CIRCLE ( 'NONE', #30294, 0.1000000000000002554 ) ;
#72138=DIRECTION ( 'NONE',  ( 0.000000000000000000, 0.000000000000000000, -1.000000000000000000 ) ) ;
#72139=DIRECTION ( 'NONE',  ( -4.274815082592931898E-19, -0.9999939076577903929, -0.003490651415223739937 ) ) ;
#72140=LINE ( 'NONE', #32873, #117836 ) ;
#72141=CIRCLE ( 'NONE', #28228, 0.1000000000000000472 ) ;
#72142=FACE_OUTER_BOUND ( 'NONE', #59979, .T. ) ;
#72143=DIRECTION ( 'NONE',  ( 0.000000000000000000, 0.000000000000000000, -1.000000000000000000 ) ) ;
#72144=AXIS2_PLACEMENT_3D ( 'NONE', #63353, #63995, #125487 ) ;
#72145=AXIS2_PLACEMENT_3D ( 'NONE', #91947, #71658, #54577 ) ;
#72147=ORIENTED_EDGE ( 'NONE', *, *, #71253, .F. ) ;
#72148=ORIENTED_EDGE ( 'NONE', *, *, #20040, .F. ) ;
#72149=CARTESIAN_POINT ( 'NONE',  ( 4.999999999999973355, 12.50000000000000000, -4.395220292106239768 ) ) ;
#72150=VERTEX_POINT ( 'NONE', #89183 ) ;
#72151=LINE ( 'NONE', #32241, #32920 ) ;
#72152=CARTESIAN_POINT ( 'NONE',  ( -8.350000000000012079, 2.500000000000000000, -1.472243186433550122 ) ) ;
#72153=VECTOR ( 'NONE', #92020, 1000.000000000000000 ) ;
#72154=CARTESIAN_POINT ( 'NONE',  ( -10.84999999999999964, 2.500000000000000000, 1.572243186433545548 ) ) ;
#72155=ORIENTED_EDGE ( 'NONE', *, *, #31543, .T. ) ;
#72156=EDGE_LOOP ( 'NONE', ( #86825, #79952 ) ) ;
#72157=EDGE_CURVE ( 'NONE', #119700, #95333, #100248, .T. ) ;
#72158=FACE_BOUND ( 'NONE', #5268, .T. ) ;
#72159=EDGE_LOOP ( 'NONE', ( #80347, #2898, #78983, #37976 ) ) ;
#72160=ADVANCED_FACE ( 'NONE', ( #110744 ), #83522, .T. ) ;
#72161=DIRECTION ( 'NONE',  ( 0.000000000000000000, 1.000000000000000000, 0.000000000000000000 ) ) ;
#72162=CARTESIAN_POINT ( 'NONE',  ( -1.650000000000034772, 12.50000000000000000, 5.802370205355744659 ) ) ;
#72163=PLANE ( 'NONE',  #103633 ) ;
#72164=DIRECTION ( 'NONE',  ( 0.000000000000000000, -0.9999939076577903929, 0.003490651415223739937 ) ) ;
#72165=DIRECTION ( 'NONE',  ( -4.274815082592931898E-19, -0.9999939076577903929, -0.003490651415223739937 ) ) ;
#72166=CARTESIAN_POINT ( 'NONE',  ( -7.499999999999980460, 12.50000000000000000, -4.330127018922201643 ) ) ;
#72167=ADVANCED_FACE ( 'NONE', ( #30922 ), #18755, .T. ) ;
#72169=EDGE_CURVE ( 'NONE', #19824, #32526, #119109, .T. ) ;
#72170=CARTESIAN_POINT ( 'NONE',  ( -8.300000000000011369, 2.500000000000000000, -0.1000000000000022815 ) ) ;
#72171=CARTESIAN_POINT ( 'NONE',  ( -14.14999999999998792, 12.50000000000000000, 2.857883832488652853 ) ) ;
#72172=FACE_OUTER_BOUND ( 'NONE', #74766, .T. ) ;
#72173=ADVANCED_FACE ( 'NONE', ( #21077 ), #81462, .T. ) ;
#72174=VECTOR ( 'NONE', #34156, 1000.000000000000000 ) ;
#72175=CARTESIAN_POINT ( 'NONE',  ( -5.650000000000023448, 12.50000000000000000, -1.753560074763288679 ) ) ;
#72176=ORIENTED_EDGE ( 'NONE', *, *, #88422, .T. ) ;
#72177=VERTEX_POINT ( 'NONE', #70190 ) ;
#72178=EDGE_LOOP ( 'NONE', ( #25651, #67101 ) ) ;
#72179=DIRECTION ( 'NONE',  ( 0.000000000000000000, 0.000000000000000000, -1.000000000000000000 ) ) ;
#72180=VERTEX_POINT ( 'NONE', #61002 ) ;
#72181=FACE_OUTER_BOUND ( 'NONE', #117950, .T. ) ;
#72182=DIRECTION ( 'NONE',  ( 0.000000000000000000, 0.000000000000000000, 1.000000000000000000 ) ) ;
#72183=ORIENTED_EDGE ( 'NONE', *, *, #69497, .T. ) ;
#72184=VERTEX_POINT ( 'NONE', #42015 ) ;
#72187=DIRECTION ( 'NONE',  ( -0.000000000000000000, -1.000000000000000000, -0.000000000000000000 ) ) ;
#72188=AXIS2_PLACEMENT_3D ( 'NONE', #33678, #73582, #14014 ) ;
#72189=CONICAL_SURFACE ( 'NONE', #22110, 0.1000000000000002554, 0.003490658503988666988 ) ;
#72190=DIRECTION ( 'NONE',  ( 0.000000000000000000, 1.000000000000000000, 0.000000000000000000 ) ) ;
#72191=FACE_OUTER_BOUND ( 'NONE', #82380, .T. ) ;
#72192=CARTESIAN_POINT ( 'NONE',  ( 9.599999999999917932, 2.500000000000000000, -0.5928203230275541635 ) ) ;
#72193=CARTESIAN_POINT ( 'NONE',  ( -12.69999999999999218, 12.50000000000000000, -4.676537180435975216 ) ) ;
#72194=DIRECTION ( 'NONE',  ( 0.000000000000000000, 1.000000000000000000, 0.000000000000000000 ) ) ;
#72195=ORIENTED_EDGE ( 'NONE', *, *, #81032, .F. ) ;
#72196=CARTESIAN_POINT ( 'NONE',  ( 6.249999999999932498, 2.500000000000000000, 5.802370205355744659 ) ) ;
#72197=ORIENTED_EDGE ( 'NONE', *, *, #101860, .F. ) ;
#72198=AXIS2_PLACEMENT_3D ( 'NONE', #9955, #91089, #100270 ) ;
#72199=VERTEX_POINT ( 'NONE', #119276 ) ;
#72200=ORIENTED_EDGE ( 'NONE', *, *, #96025, .F. ) ;
#72201=AXIS2_PLACEMENT_3D ( 'NONE', #74398, #43671, #54739 ) ;
#72202=LINE ( 'NONE', #112121, #12948 ) ;
#72203=VERTEX_POINT ( 'NONE', #90450 ) ;
#72204=ORIENTED_EDGE ( 'NONE', *, *, #110458, .T. ) ;
#72205=ORIENTED_EDGE ( 'NONE', *, *, #55096, .F. ) ;
#72206=DIRECTION ( 'NONE',  ( -0.000000000000000000, 1.000000000000000000, -0.000000000000000000 ) ) ;
#72207=DIRECTION ( 'NONE',  ( -0.000000000000000000, 1.000000000000000000, -0.000000000000000000 ) ) ;
#72208=CONICAL_SURFACE ( 'NONE', #47071, 0.1000000000000002554, 0.003490658503988666988 ) ;
#72209=CARTESIAN_POINT ( 'NONE',  ( 6.249999999999930722, 12.50000000000000000, 7.188010851410848723 ) ) ;
#72210=CARTESIAN_POINT ( 'NONE',  ( -11.69999999999999929, 12.50000000000000000, -4.395220292106237103 ) ) ;
#72211=DIRECTION ( 'NONE',  ( 0.000000000000000000, -0.000000000000000000, 1.000000000000000000 ) ) ;
#72212=EDGE_CURVE ( 'NONE', #115792, #31757, #81925, .T. ) ;
#72213=DIRECTION ( 'NONE',  ( 0.000000000000000000, 0.000000000000000000, 1.000000000000000000 ) ) ;
#72214=EDGE_CURVE ( 'NONE', #123959, #20030, #4085, .T. ) ;
#72215=EDGE_CURVE ( 'NONE', #88410, #42865, #13937, .T. ) ;
#72216=CARTESIAN_POINT ( 'NONE',  ( -2.900000000000030553, 2.500000000000000000, 5.122947341949749323 ) ) ;
#72217=VERTEX_POINT ( 'NONE', #109466 ) ;
#72218=LINE ( 'NONE', #3464, #42104 ) ;
#72219=EDGE_LOOP ( 'NONE', ( #123243, #116350 ) ) ;
#72220=DIRECTION ( 'NONE',  ( 0.000000000000000000, -0.000000000000000000, 1.000000000000000000 ) ) ;
#72221=VECTOR ( 'NONE', #69250, 1000.000000000000000 ) ;
#72222=EDGE_CURVE ( 'NONE', #63429, #102522, #9977, .T. ) ;
#72223=EDGE_LOOP ( 'NONE', ( #45845, #116192, #87606, #96042 ) ) ;
#72224=CARTESIAN_POINT ( 'NONE',  ( 4.399999999999939071, 2.500000000000000000, -0.3464101615137782364 ) ) ;
#72225=ADVANCED_FACE ( 'NONE', ( #89820 ), #116943, .T. ) ;
#72226=AXIS2_PLACEMENT_3D ( 'NONE', #78490, #79127, #76541 ) ;
#72227=ORIENTED_EDGE ( 'NONE', *, *, #4945, .F. ) ;
#72228=EDGE_CURVE ( 'NONE', #99657, #107914, #110112, .T. ) ;
#72229=DIRECTION ( 'NONE',  ( 0.000000000000000000, 0.000000000000000000, 1.000000000000000000 ) ) ;
#72230=ADVANCED_FACE ( 'NONE', ( #34791 ), #104434, .T. ) ;
#72231=ADVANCED_FACE ( 'NONE', ( #2722 ), #79417, .T. ) ;
#72232=AXIS2_PLACEMENT_3D ( 'NONE', #73178, #94104, #2483 ) ;
#72233=CARTESIAN_POINT ( 'NONE',  ( -3.150000000000033218, 12.50000000000000000, -6.776507416713040577 ) ) ;
#72234=EDGE_LOOP ( 'NONE', ( #82461, #128330, #114156, #49473 ) ) ;
#72235=ORIENTED_EDGE ( 'NONE', *, *, #13510, .F. ) ;
#72236=CARTESIAN_POINT ( 'NONE',  ( 9.599999999999917932, 2.500000000000000000, 0.6928203230275494784 ) ) ;
#72237=DIRECTION ( 'NONE',  ( 0.000000000000000000, 0.000000000000000000, 1.000000000000000000 ) ) ;
#72238=LINE ( 'NONE', #84622, #18801 ) ;
#72239=CARTESIAN_POINT ( 'NONE',  ( 8.349999999999923261, 12.50000000000000000, -6.495190528383302464 ) ) ;
#72240=EDGE_CURVE ( 'NONE', #11992, #100514, #112852, .T. ) ;
#72241=CONICAL_SURFACE ( 'NONE', #101471, 0.1000000000000000472, 0.003490658503988666988 ) ;
#72242=FACE_OUTER_BOUND ( 'NONE', #21790, .T. ) ;
#72243=AXIS2_PLACEMENT_3D ( 'NONE', #111769, #11625, #122245 ) ;
#72244=ORIENTED_EDGE ( 'NONE', *, *, #17145, .T. ) ;
#72245=AXIS2_PLACEMENT_3D ( 'NONE', #55780, #26332, #66235 ) ;
#72246=CARTESIAN_POINT ( 'NONE',  ( 2.500000000000002220, -2.500000000000000000, -8.999999999999998224 ) ) ;
#72247=CONICAL_SURFACE ( 'NONE', #124457, 0.09999999999999982514, 0.003490658503988666988 ) ;
#72248=ORIENTED_EDGE ( 'NONE', *, *, #52274, .T. ) ;
#72250=DIRECTION ( 'NONE',  ( 0.000000000000000000, 0.000000000000000000, -1.000000000000000000 ) ) ;
#72251=AXIS2_PLACEMENT_3D ( 'NONE', #106905, #27075, #35611 ) ;
#72252=VECTOR ( 'NONE', #26461, 1000.000000000000000 ) ;
#72253=CONICAL_SURFACE ( 'NONE', #95231, 0.1000000000000002554, 0.003490658503988666988 ) ;
#72254=CARTESIAN_POINT ( 'NONE',  ( 6.849999999999927702, 2.500000000000000000, 1.818653347947321475 ) ) ;
#72255=FACE_OUTER_BOUND ( 'NONE', #35699, .T. ) ;
#72256=DIRECTION ( 'NONE',  ( -0.000000000000000000, -1.000000000000000000, -0.000000000000000000 ) ) ;
#72257=DIRECTION ( 'NONE',  ( 0.000000000000000000, 0.000000000000000000, 1.000000000000000000 ) ) ;
#72258=DIRECTION ( 'NONE',  ( 0.000000000000000000, 0.000000000000000000, 1.000000000000000000 ) ) ;
#72259=ORIENTED_EDGE ( 'NONE', *, *, #128966, .F. ) ;
#72260=PLANE ( 'NONE',  #25002 ) ;
#72261=FACE_OUTER_BOUND ( 'NONE', #117170, .T. ) ;
#72262=DIRECTION ( 'NONE',  ( -0.000000000000000000, 1.000000000000000000, -0.000000000000000000 ) ) ;
#72263=ORIENTED_EDGE ( 'NONE', *, *, #20914, .F. ) ;
#72264=ORIENTED_EDGE ( 'NONE', *, *, #119268, .T. ) ;
#72265=DIRECTION ( 'NONE',  ( 0.000000000000000000, 1.000000000000000000, 0.000000000000000000 ) ) ;
#72266=EDGE_CURVE ( 'NONE', #87169, #85514, #58494, .T. ) ;
#72267=ORIENTED_EDGE ( 'NONE', *, *, #47822, .T. ) ;
#72269=ORIENTED_EDGE ( 'NONE', *, *, #7719, .F. ) ;
#72270=CARTESIAN_POINT ( 'NONE',  ( -4.400000000000028777, 2.500000000000000000, -4.676537180435978769 ) ) ;
#72271=CONICAL_SURFACE ( 'NONE', #109922, 0.09999999999999982514, 0.003490658503988666988 ) ;
#72272=ORIENTED_EDGE ( 'NONE', *, *, #77041, .F. ) ;
#72273=CARTESIAN_POINT ( 'NONE',  ( 16.58100817949905803, -2.557139044001862427, -6.067820687739756025 ) ) ;
#72274=CARTESIAN_POINT ( 'NONE',  ( -9.150000000000009237, 2.500000000000000000, 2.857883832488649301 ) ) ;
#72275=CARTESIAN_POINT ( 'NONE',  ( 16.53754090007008415, 0.4856821978169202358, 6.114873053042321871 ) ) ;
#72276=CIRCLE ( 'NONE', #24148, 0.1000000000000000472 ) ;
#72277=CONICAL_SURFACE ( 'NONE', #78637, 0.1000000000000002554, 0.003490658503988666988 ) ;
#72278=EDGE_LOOP ( 'NONE', ( #50671, #83693 ) ) ;
#72279=DIRECTION ( 'NONE',  ( 0.000000000000000000, 0.000000000000000000, 1.000000000000000000 ) ) ;
#72280=CARTESIAN_POINT ( 'NONE',  ( -5.200000000000022382, 2.500000000000000000, 0.4464101615137735513 ) ) ;
#72281=ADVANCED_FACE ( 'NONE', ( #123775 ), #75193, .T. ) ;
#72282=VERTEX_POINT ( 'NONE', #124444 ) ;
#72283=CIRCLE ( 'NONE', #34642, 0.06509327318403745899 ) ;
#72284=ORIENTED_EDGE ( 'NONE', *, *, #106281, .F. ) ;
#72285=AXIS2_PLACEMENT_3D ( 'NONE', #57496, #97409, #7728 ) ;
#72286=ORIENTED_EDGE ( 'NONE', *, *, #73924, .T. ) ;
#72287=FACE_OUTER_BOUND ( 'NONE', #17282, .T. ) ;
#72289=PLANE ( 'NONE',  #102750 ) ;
#72290=FACE_BOUND ( 'NONE', #103872, .T. ) ;
#72291=ORIENTED_EDGE ( 'NONE', *, *, #47576, .T. ) ;
#72292=CARTESIAN_POINT ( 'NONE',  ( 5.199999999999937117, 12.50000000000000000, -4.676537180435978769 ) ) ;
#72293=DIRECTION ( 'NONE',  ( 0.000000000000000000, 0.000000000000000000, 1.000000000000000000 ) ) ;
#72294=ORIENTED_EDGE ( 'NONE', *, *, #36207, .F. ) ;
#72295=DIRECTION ( 'NONE',  ( -0.000000000000000000, -1.000000000000000000, -0.000000000000000000 ) ) ;
#72296=AXIS2_PLACEMENT_3D ( 'NONE', #43482, #103021, #13347 ) ;
#72297=DIRECTION ( 'NONE',  ( 0.000000000000000000, 0.000000000000000000, 1.000000000000000000 ) ) ;
#72298=AXIS2_PLACEMENT_3D ( 'NONE', #56368, #34173, #4669 ) ;
#72299=PLANE ( 'NONE',  #75769 ) ;
#72300=DIRECTION ( 'NONE',  ( 0.000000000000000000, 0.000000000000000000, -1.000000000000000000 ) ) ;
#72301=CARTESIAN_POINT ( 'NONE',  ( -8.750000000000010658, 2.500000000000000000, 2.957883832488649389 ) ) ;
#72302=DIRECTION ( 'NONE',  ( 0.000000000000000000, -0.9999939076577903929, 0.003490651415223739937 ) ) ;
#72303=DIRECTION ( 'NONE',  ( 0.000000000000000000, 0.000000000000000000, 1.000000000000000000 ) ) ;
#72304=EDGE_CURVE ( 'NONE', #72798, #52727, #84517, .T. ) ;
#72305=VERTEX_POINT ( 'NONE', #34138 ) ;
#72306=EDGE_LOOP ( 'NONE', ( #97748, #37962, #6786, #66053 ) ) ;
#72307=ORIENTED_EDGE ( 'NONE', *, *, #16166, .T. ) ;
#72308=VERTEX_POINT ( 'NONE', #55059 ) ;
#72309=DIRECTION ( 'NONE',  ( 0.000000000000000000, 1.000000000000000000, 0.000000000000000000 ) ) ;
#72310=DIRECTION ( 'NONE',  ( -4.274815082592931898E-19, -0.9999939076577903929, -0.003490651415223739937 ) ) ;
#72311=DIRECTION ( 'NONE',  ( 0.000000000000000000, 0.000000000000000000, 1.000000000000000000 ) ) ;
#72312=ORIENTED_EDGE ( 'NONE', *, *, #123740, .T. ) ;
#72313=FACE_BOUND ( 'NONE', #44187, .T. ) ;
#72314=ADVANCED_FACE ( 'NONE', ( #45244 ), #106578, .T. ) ;
#72315=DIRECTION ( 'NONE',  ( 0.000000000000000000, 1.000000000000000000, 0.000000000000000000 ) ) ;
#72316=CARTESIAN_POINT ( 'NONE',  ( 2.499999999999948930, 2.500000000000000000, -0.6928203230275541413 ) ) ;
#72317=CARTESIAN_POINT ( 'NONE',  ( -6.650000000000014566, 12.50000000000000000, 1.407149913249508000 ) ) ;
#72318=CIRCLE ( 'NONE', #3259, 0.06509327318403745899 ) ;
#72319=DIRECTION ( 'NONE',  ( -0.000000000000000000, -1.000000000000000000, -0.000000000000000000 ) ) ;
#72320=CIRCLE ( 'NONE', #122487, 0.1000000000000002554 ) ;
#72321=DIRECTION ( 'NONE',  ( 0.000000000000000000, 0.000000000000000000, 1.000000000000000000 ) ) ;
#72323=CARTESIAN_POINT ( 'NONE',  ( 1.049999999999954969, 12.50000000000000000, -6.841600689897077814 ) ) ;
#72324=EDGE_CURVE ( 'NONE', #99720, #113921, #54267, .T. ) ;
#72325=DIRECTION ( 'NONE',  ( 0.000000000000000000, 0.000000000000000000, 1.000000000000000000 ) ) ;
#72326=DIRECTION ( 'NONE',  ( -0.000000000000000000, -1.000000000000000000, -0.000000000000000000 ) ) ;
#72327=EDGE_CURVE ( 'NONE', #8589, #83800, #43822, .T. ) ;
#72328=FACE_OUTER_BOUND ( 'NONE', #98391, .T. ) ;
#72329=ADVANCED_FACE ( 'NONE', ( #33502 ), #73142, .T. ) ;
#72330=ADVANCED_FACE ( 'NONE', ( #63594 ), #27084, .T. ) ;
#72331=EDGE_LOOP ( 'NONE', ( #129518, #126634, #99837, #35430 ) ) ;
#72332=EDGE_LOOP ( 'NONE', ( #72432, #113867 ) ) ;
#72333=ORIENTED_EDGE ( 'NONE', *, *, #15560, .F. ) ;
#72334=EDGE_LOOP ( 'NONE', ( #18635, #44395, #9083, #52045 ) ) ;
#72335=EDGE_LOOP ( 'NONE', ( #5861, #42962, #96337, #120709 ) ) ;
#72336=ORIENTED_EDGE ( 'NONE', *, *, #50360, .T. ) ;
#72337=VECTOR ( 'NONE', #19257, 1000.000000000000000 ) ;
#72339=ORIENTED_EDGE ( 'NONE', *, *, #122118, .T. ) ;
#72340=ADVANCED_FACE ( 'NONE', ( #113978 ), #6301, .T. ) ;
#72341=VERTEX_POINT ( 'NONE', #82596 ) ;
#72342=EDGE_CURVE ( 'NONE', #102565, #40749, #122513, .T. ) ;
#72343=AXIS2_PLACEMENT_3D ( 'NONE', #11930, #32250, #102883 ) ;
#72344=EDGE_CURVE ( 'NONE', #121499, #49607, #102849, .T. ) ;
#72345=CARTESIAN_POINT ( 'NONE',  ( -4.200000000000025935, 2.500000000000000000, 4.330127018922196314 ) ) ;
#72346=DIRECTION ( 'NONE',  ( 0.000000000000000000, 0.000000000000000000, 1.000000000000000000 ) ) ;
#72347=CARTESIAN_POINT ( 'NONE',  ( -5.850000000000021849, 12.50000000000000000, -1.537336459617587581 ) ) ;
#72348=DIRECTION ( 'NONE',  ( 0.000000000000000000, 0.000000000000000000, 1.000000000000000000 ) ) ;
#72349=AXIS2_PLACEMENT_3D ( 'NONE', #71925, #61464, #31356 ) ;
#72350=ORIENTED_EDGE ( 'NONE', *, *, #55551, .T. ) ;
#72352=VERTEX_POINT ( 'NONE', #73397 ) ;
#72353=ORIENTED_EDGE ( 'NONE', *, *, #45455, .F. ) ;
#72354=DIRECTION ( 'NONE',  ( 0.000000000000000000, 1.000000000000000000, 0.000000000000000000 ) ) ;
#72355=DIRECTION ( 'NONE',  ( 0.000000000000000000, 0.000000000000000000, 1.000000000000000000 ) ) ;
#72356=VECTOR ( 'NONE', #95493, 1000.000000000000000 ) ;
#72357=EDGE_LOOP ( 'NONE', ( #106506, #93131 ) ) ;
#72358=EDGE_LOOP ( 'NONE', ( #23287, #30588 ) ) ;
#72359=CARTESIAN_POINT ( 'NONE',  ( 7.299999999999927880, 2.500000000000000000, -4.776537180435977525 ) ) ;
#72360=CARTESIAN_POINT ( 'NONE',  ( 10.84999999999990905, 12.50000000000000000, -7.253104124594891289 ) ) ;
#72361=CARTESIAN_POINT ( 'NONE',  ( -3.750000000000025757, 2.500000000000000000, 1.472243186433545459 ) ) ;
#72362=FACE_OUTER_BOUND ( 'NONE', #23327, .T. ) ;
#72363=CARTESIAN_POINT ( 'NONE',  ( 3.549999999999942091, 2.500000000000000000, 2.411473670974873862 ) ) ;
#72364=VECTOR ( 'NONE', #94207, 1000.000000000000000 ) ;
#72365=AXIS2_PLACEMENT_3D ( 'NONE', #62950, #61013, #81312 ) ;
#72366=EDGE_LOOP ( 'NONE', ( #61358, #54539, #22424, #115259 ) ) ;
#72367=ADVANCED_FACE ( 'NONE', ( #83240 ), #93693, .T. ) ;
#72368=CARTESIAN_POINT ( 'NONE',  ( 7.499999999999925393, 12.50000000000000000, -0.6928203230275541413 ) ) ;
#72369=VECTOR ( 'NONE', #114777, 1000.000000000000000 ) ;
#72370=EDGE_LOOP ( 'NONE', ( #115407, #36765, #32316, #118345 ) ) ;
#72371=AXIS2_PLACEMENT_3D ( 'NONE', #59599, #101428, #80511 ) ;
#72372=CARTESIAN_POINT ( 'NONE',  ( 17.50000000000000000, 2.499999999999999556, 0.6666666666666699603 ) ) ;
#72373=EDGE_CURVE ( 'NONE', #58339, #39516, #89945, .T. ) ;
#72374=DIRECTION ( 'NONE',  ( 0.000000000000000000, 0.000000000000000000, 1.000000000000000000 ) ) ;
#72375=DIRECTION ( 'NONE',  ( 0.000000000000000000, 0.000000000000000000, 1.000000000000000000 ) ) ;
#72376=PLANE ( 'NONE',  #15183 ) ;
#72377=EDGE_CURVE ( 'NONE', #3400, #54303, #18842, .T. ) ;
#72378=DIRECTION ( 'NONE',  ( -0.000000000000000000, -1.000000000000000000, -0.000000000000000000 ) ) ;
#72379=ORIENTED_EDGE ( 'NONE', *, *, #99833, .F. ) ;
#72380=AXIS2_PLACEMENT_3D ( 'NONE', #73875, #3842, #113809 ) ;
#72381=EDGE_CURVE ( 'NONE', #12969, #40542, #8372, .T. ) ;
#72382=CARTESIAN_POINT ( 'NONE',  ( 5.449999999999934452, 2.500000000000000000, 2.065063509461097624 ) ) ;
#72383=CONICAL_SURFACE ( 'NONE', #126658, 0.1000000000000002554, 0.003490658503988666988 ) ;
#72384=VECTOR ( 'NONE', #78284, 1000.000000000000000 ) ;
#72385=EDGE_CURVE ( 'NONE', #70518, #67980, #119608, .T. ) ;
#72386=CARTESIAN_POINT ( 'NONE',  ( -12.69999999999999396, 2.500000000000000000, -3.883716857408423984 ) ) ;
#72387=ORIENTED_EDGE ( 'NONE', *, *, #59381, .F. ) ;
#72388=ORIENTED_EDGE ( 'NONE', *, *, #6821, .F. ) ;
#72389=ORIENTED_EDGE ( 'NONE', *, *, #11631, .F. ) ;
#72390=CARTESIAN_POINT ( 'NONE',  ( -4.550000000000022915, 2.500000000000000000, -2.165063509461101710 ) ) ;
#72391=CARTESIAN_POINT ( 'NONE',  ( 8.949999999999921130, 12.50000000000000000, 1.753560074763284016 ) ) ;
#72393=CARTESIAN_POINT ( 'NONE',  ( -11.64999999999999680, 12.50000000000000000, 7.188010851410848723 ) ) ;
#72394=EDGE_CURVE ( 'NONE', #3125, #60519, #39803, .T. ) ;
#72395=DIRECTION ( 'NONE',  ( 0.000000000000000000, 1.000000000000000000, 0.000000000000000000 ) ) ;
#72396=CARTESIAN_POINT ( 'NONE',  ( 16.68631762705676636, 1.607367762582524451, -5.954228785333302021 ) ) ;
#72397=DIRECTION ( 'NONE',  ( 0.000000000000000000, 1.000000000000000000, 0.000000000000000000 ) ) ;
#72398=CARTESIAN_POINT ( 'NONE',  ( 11.89999999999990798, 12.50000000000000000, -4.676537180435977881 ) ) ;
#72399=VERTEX_POINT ( 'NONE', #69878 ) ;
#72400=LINE ( 'NONE', #22657, #46388 ) ;
#72401=DIRECTION ( 'NONE',  ( 0.000000000000000000, -0.000000000000000000, 1.000000000000000000 ) ) ;
#72402=EDGE_CURVE ( 'NONE', #36233, #99874, #112945, .T. ) ;
#72403=DIRECTION ( 'NONE',  ( 0.000000000000000000, 0.000000000000000000, -1.000000000000000000 ) ) ;
#72404=DIRECTION ( 'NONE',  ( 0.000000000000000000, -0.000000000000000000, -1.000000000000000000 ) ) ;
#72405=ORIENTED_EDGE ( 'NONE', *, *, #42146, .F. ) ;
#72406=DIRECTION ( 'NONE',  ( -0.000000000000000000, -1.000000000000000000, -0.000000000000000000 ) ) ;
#72407=AXIS2_PLACEMENT_3D ( 'NONE', #38771, #28935, #29562 ) ;
#72408=DIRECTION ( 'NONE',  ( -0.000000000000000000, -1.000000000000000000, -0.000000000000000000 ) ) ;
#72409=DIRECTION ( 'NONE',  ( 0.000000000000000000, 1.000000000000000000, 0.000000000000000000 ) ) ;
#72410=ORIENTED_EDGE ( 'NONE', *, *, #64156, .T. ) ;
#72411=VERTEX_POINT ( 'NONE', #108501 ) ;
#72412=AXIS2_PLACEMENT_3D ( 'NONE', #49884, #108, #40050 ) ;
#72413=AXIS2_PLACEMENT_3D ( 'NONE', #80979, #81612, #29953 ) ;
#72414=LINE ( 'NONE', #69827, #65637 ) ;
#72415=EDGE_CURVE ( 'NONE', #83060, #56205, #35584, .T. ) ;
#72416=ORIENTED_EDGE ( 'NONE', *, *, #37782, .T. ) ;
#72417=EDGE_LOOP ( 'NONE', ( #5668, #49167 ) ) ;
#72418=DIRECTION ( 'NONE',  ( -0.000000000000000000, 1.000000000000000000, -0.000000000000000000 ) ) ;
#72419=DIRECTION ( 'NONE',  ( -0.000000000000000000, 1.000000000000000000, -0.000000000000000000 ) ) ;
#72420=CARTESIAN_POINT ( 'NONE',  ( -12.49999999999999289, 2.500000000000000000, 3.737306695894644371 ) ) ;
#72421=CIRCLE ( 'NONE', #84931, 0.06509327318403745899 ) ;
#72422=CIRCLE ( 'NONE', #43187, 0.1000000000000000472 ) ;
#72423=CARTESIAN_POINT ( 'NONE',  ( 13.29999999999990301, 2.500000000000000000, -4.330127018922201643 ) ) ;
#72424=EDGE_LOOP ( 'NONE', ( #112793, #38666, #61743, #9166 ) ) ;
#72425=AXIS2_PLACEMENT_3D ( 'NONE', #36627, #76538, #16297 ) ;
#72426=DIRECTION ( 'NONE',  ( 0.000000000000000000, 1.000000000000000000, 0.000000000000000000 ) ) ;
#72427=VERTEX_POINT ( 'NONE', #58769 ) ;
#72428=DIRECTION ( 'NONE',  ( 0.000000000000000000, 0.000000000000000000, -1.000000000000000000 ) ) ;
#72429=EDGE_CURVE ( 'NONE', #14821, #78690, #56488, .T. ) ;
#72430=FACE_OUTER_BOUND ( 'NONE', #52337, .T. ) ;
#72431=ORIENTED_EDGE ( 'NONE', *, *, #104508, .F. ) ;
#72432=ORIENTED_EDGE ( 'NONE', *, *, #96035, .T. ) ;
#72433=ORIENTED_EDGE ( 'NONE', *, *, #70847, .F. ) ;
#72434=VERTEX_POINT ( 'NONE', #49609 ) ;
#72435=DIRECTION ( 'NONE',  ( 0.000000000000000000, 0.000000000000000000, -1.000000000000000000 ) ) ;
#72436=CARTESIAN_POINT ( 'NONE',  ( 13.80679872386854790, 1.500000000000063727, 7.946844943073665846 ) ) ;
#72437=DIRECTION ( 'NONE',  ( -0.000000000000000000, -1.000000000000000000, -0.000000000000000000 ) ) ;
#72438=FACE_BOUND ( 'NONE', #103867, .T. ) ;
#72439=ORIENTED_EDGE ( 'NONE', *, *, #116543, .T. ) ;
#72440=AXIS2_PLACEMENT_3D ( 'NONE', #68601, #67956, #50266 ) ;
#72442=DIRECTION ( 'NONE',  ( 0.000000000000000000, 1.000000000000000000, 0.000000000000000000 ) ) ;
#72443=DIRECTION ( 'NONE',  ( 0.000000000000000000, 0.000000000000000000, 1.000000000000000000 ) ) ;
#72444=VECTOR ( 'NONE', #281, 1000.000000000000000 ) ;
#72446=CONICAL_SURFACE ( 'NONE', #126859, 0.09999999999999982514, 0.003490658503988666988 ) ;
#72447=CARTESIAN_POINT ( 'NONE',  ( -10.40000000000000213, 12.50000000000000000, 4.265033745738159077 ) ) ;
#72448=FACE_OUTER_BOUND ( 'NONE', #73128, .T. ) ;
#72449=AXIS2_PLACEMENT_3D ( 'NONE', #24317, #98680, #9014 ) ;
#72450=AXIS2_PLACEMENT_3D ( 'NONE', #57808, #98354, #59098 ) ;
#72451=DIRECTION ( 'NONE',  ( 0.000000000000000000, 0.000000000000000000, -1.000000000000000000 ) ) ;
#72452=AXIS2_PLACEMENT_3D ( 'NONE', #22880, #62800, #62164 ) ;
#72453=EDGE_CURVE ( 'NONE', #71159, #16443, #110784, .T. ) ;
#72454=ORIENTED_EDGE ( 'NONE', *, *, #70117, .T. ) ;
#72455=ORIENTED_EDGE ( 'NONE', *, *, #61064, .F. ) ;
#72456=VERTEX_POINT ( 'NONE', #115227 ) ;
#72457=VERTEX_POINT ( 'NONE', #96251 ) ;
#72458=VERTEX_POINT ( 'NONE', #95630 ) ;
#72459=DIRECTION ( 'NONE',  ( 0.000000000000000000, 0.000000000000000000, 1.000000000000000000 ) ) ;
#72460=CARTESIAN_POINT ( 'NONE',  ( 8.949999999999917577, 2.500000000000000000, -2.411473670974877859 ) ) ;
#72461=VERTEX_POINT ( 'NONE', #90135 ) ;
#72462=FACE_BOUND ( 'NONE', #19999, .T. ) ;
#72463=CIRCLE ( 'NONE', #89276, 0.06509327318403745899 ) ;
#72464=DIRECTION ( 'NONE',  ( 0.000000000000000000, 0.000000000000000000, 1.000000000000000000 ) ) ;
#72465=ADVANCED_FACE ( 'NONE', ( #20131 ), #94069, .T. ) ;
#72466=AXIS2_PLACEMENT_3D ( 'NONE', #32609, #73149, #52223 ) ;
#72467=ORIENTED_EDGE ( 'NONE', *, *, #22987, .T. ) ;
#72468=EDGE_CURVE ( 'NONE', #74932, #16115, #100336, .T. ) ;
#72469=DIRECTION ( 'NONE',  ( 0.000000000000000000, 0.000000000000000000, 1.000000000000000000 ) ) ;
#72470=ADVANCED_FACE ( 'NONE', ( #106093 ), #69013, .T. ) ;
#72471=DIRECTION ( 'NONE',  ( 0.000000000000000000, 1.000000000000000000, 0.000000000000000000 ) ) ;
#72472=ADVANCED_FACE ( 'NONE', ( #25577 ), #85740, .T. ) ;
#72473=DIRECTION ( 'NONE',  ( 0.000000000000000000, 1.000000000000000000, 0.000000000000000000 ) ) ;
#72474=ADVANCED_FACE ( 'NONE', ( #5931 ), #73235, .T. ) ;
#72475=ORIENTED_EDGE ( 'NONE', *, *, #89326, .F. ) ;
#72476=DIRECTION ( 'NONE',  ( -4.274815082592931898E-19, -0.9999939076577903929, -0.003490651415223739937 ) ) ;
#72477=ORIENTED_EDGE ( 'NONE', *, *, #119160, .T. ) ;
#72478=EDGE_LOOP ( 'NONE', ( #114654, #64912, #88464, #94532 ) ) ;
#72479=EDGE_CURVE ( 'NONE', #92776, #73985, #46049, .T. ) ;
#72480=ORIENTED_EDGE ( 'NONE', *, *, #126989, .F. ) ;
#72481=CARTESIAN_POINT ( 'NONE',  ( -11.25000000000000000, 12.50000000000000000, 2.857883832488649301 ) ) ;
#72482=EDGE_CURVE ( 'NONE', #112003, #92128, #98673, .T. ) ;
#72484=DIRECTION ( 'NONE',  ( 0.000000000000000000, 0.000000000000000000, 1.000000000000000000 ) ) ;
#72485=VERTEX_POINT ( 'NONE', #29313 ) ;
#72486=EDGE_CURVE ( 'NONE', #896, #120378, #62, .T. ) ;
#72487=CARTESIAN_POINT ( 'NONE',  ( 0.5999999999999621192, 2.500000000000000000, 0.2464101615137758439 ) ) ;
#72488=ADVANCED_FACE ( 'NONE', ( #111059 ), #110435, .T. ) ;
#72489=DIRECTION ( 'NONE',  ( 0.000000000000000000, 0.000000000000000000, 1.000000000000000000 ) ) ;
#72490=EDGE_CURVE ( 'NONE', #60519, #3125, #16766, .T. ) ;
#72491=FACE_OUTER_BOUND ( 'NONE', #35641, .T. ) ;
#72492=CARTESIAN_POINT ( 'NONE',  ( -9.150000000000009237, 12.50000000000000000, -2.099970236277064473 ) ) ;
#72494=VERTEX_POINT ( 'NONE', #22726 ) ;
#72495=PLANE ( 'NONE',  #64150 ) ;
#72497=EDGE_LOOP ( 'NONE', ( #8574, #59769 ) ) ;
#72498=DIRECTION ( 'NONE',  ( 0.000000000000000000, 0.000000000000000000, -1.000000000000000000 ) ) ;
#72499=AXIS2_PLACEMENT_3D ( 'NONE', #22281, #29507, #62203 ) ;
#72500=EDGE_LOOP ( 'NONE', ( #128625, #118007, #53779, #51954 ) ) ;
#72501=CIRCLE ( 'NONE', #110055, 0.06509327318403745899 ) ;
#72502=ORIENTED_EDGE ( 'NONE', *, *, #62288, .F. ) ;
#72503=PLANE ( 'NONE',  #30459 ) ;
#72504=DIRECTION ( 'NONE',  ( 0.000000000000000000, 1.000000000000000000, 0.000000000000000000 ) ) ;
#72505=DIRECTION ( 'NONE',  ( 0.000000000000000000, 1.000000000000000000, 0.000000000000000000 ) ) ;
#72506=CARTESIAN_POINT ( 'NONE',  ( 12.89999999999990088, 2.500000000000000000, -4.430127018922202176 ) ) ;
#72507=FACE_OUTER_BOUND ( 'NONE', #71872, .T. ) ;
#72508=EDGE_LOOP ( 'NONE', ( #91267, #111889, #107261, #44914 ) ) ;
#72509=AXIS2_PLACEMENT_3D ( 'NONE', #64186, #34753, #53728 ) ;
#72510=VECTOR ( 'NONE', #54093, 1000.000000000000000 ) ;
#72511=ORIENTED_EDGE ( 'NONE', *, *, #24651, .F. ) ;
#72512=CARTESIAN_POINT ( 'NONE',  ( 9.999999999999911182, 2.500000000000000000, 5.022947341949748790 ) ) ;
#72513=DIRECTION ( 'NONE',  ( 0.000000000000000000, 0.000000000000000000, 1.000000000000000000 ) ) ;
#72514=DIRECTION ( 'NONE',  ( 0.000000000000000000, 0.000000000000000000, 1.000000000000000000 ) ) ;
#72515=ORIENTED_EDGE ( 'NONE', *, *, #98731, .T. ) ;
#72516=ORIENTED_EDGE ( 'NONE', *, *, #103795, .F. ) ;
#72517=AXIS2_PLACEMENT_3D ( 'NONE', #76019, #104814, #95026 ) ;
#72518=LINE ( 'NONE', #126110, #16379 ) ;
#72519=AXIS2_PLACEMENT_3D ( 'NONE', #20391, #31497, #49226 ) ;
#72520=VECTOR ( 'NONE', #10452, 1000.000000000000000 ) ;
#72521=ORIENTED_EDGE ( 'NONE', *, *, #83900, .T. ) ;
#72522=LINE ( 'NONE', #60555, #102976 ) ;
#72523=DIRECTION ( 'NONE',  ( 0.000000000000000000, 0.000000000000000000, 1.000000000000000000 ) ) ;
#72524=CONICAL_SURFACE ( 'NONE', #105954, 0.1000000000000000472, 0.003490658503988666988 ) ;
#72525=LINE ( 'NONE', #3134, #76252 ) ;
#72526=ORIENTED_EDGE ( 'NONE', *, *, #67428, .T. ) ;
#72527=PLANE ( 'NONE',  #14696 ) ;
#72528=CARTESIAN_POINT ( 'NONE',  ( -7.900000000000014566, 12.50000000000000000, -4.330127018922201643 ) ) ;
#72529=CARTESIAN_POINT ( 'NONE',  ( -5.800000000000018474, 2.500000000000000000, 0.09999999999999772959 ) ) ;
#72530=DIRECTION ( 'NONE',  ( 0.000000000000000000, 1.000000000000000000, 0.000000000000000000 ) ) ;
#72531=DIRECTION ( 'NONE',  ( 0.000000000000000000, -0.000000000000000000, 1.000000000000000000 ) ) ;
#72532=ORIENTED_EDGE ( 'NONE', *, *, #31383, .F. ) ;
#72533=EDGE_CURVE ( 'NONE', #10550, #40796, #27162, .T. ) ;
#72534=CARTESIAN_POINT ( 'NONE',  ( 97.50000000000000000, 9.184850993605147944E-16, -7.500000000000000000 ) ) ;
#72535=CARTESIAN_POINT ( 'NONE',  ( 9.999999999999948486, 12.50000000000000000, 4.330127018922196314 ) ) ;
#72536=EDGE_CURVE ( 'NONE', #90750, #75566, #50254, .T. ) ;
#72537=ORIENTED_EDGE ( 'NONE', *, *, #106725, .F. ) ;
#72538=ORIENTED_EDGE ( 'NONE', *, *, #70404, .T. ) ;
#72540=CARTESIAN_POINT ( 'NONE',  ( 13.29999999999990301, 2.500000000000000000, -4.230127018922201998 ) ) ;
#72541=CIRCLE ( 'NONE', #124754, 0.06509327318403745899 ) ;
#72542=CARTESIAN_POINT ( 'NONE',  ( 0.1999999999999571565, 12.50000000000000000, 4.048810130592458201 ) ) ;
#72544=DIRECTION ( 'NONE',  ( 0.000000000000000000, 0.000000000000000000, 1.000000000000000000 ) ) ;
#72546=EDGE_CURVE ( 'NONE', #101260, #22692, #123306, .T. ) ;
#72547=CARTESIAN_POINT ( 'NONE',  ( 2.299999999999949640, 2.500000000000000000, -4.776537180435977525 ) ) ;
#72548=DIRECTION ( 'NONE',  ( 0.000000000000000000, 0.000000000000000000, -1.000000000000000000 ) ) ;
#72549=AXIS2_PLACEMENT_3D ( 'NONE', #43466, #50685, #83383 ) ;
#72550=DIRECTION ( 'NONE',  ( 0.000000000000000000, 0.000000000000000000, 1.000000000000000000 ) ) ;
#72551=LINE ( 'NONE', #62729, #62343 ) ;
#72552=AXIS2_PLACEMENT_3D ( 'NONE', #109147, #128170, #120282 ) ;
#72553=CARTESIAN_POINT ( 'NONE',  ( -6.850000000000013856, 2.500000000000000000, 6.941600689897073018 ) ) ;
#72554=ORIENTED_EDGE ( 'NONE', *, *, #88419, .F. ) ;
#72555=EDGE_LOOP ( 'NONE', ( #18898, #79346 ) ) ;
#72556=AXIS2_PLACEMENT_3D ( 'NONE', #78701, #68855, #59048 ) ;
#72557=EDGE_LOOP ( 'NONE', ( #22120, #96688, #125584, #9873 ) ) ;
#72558=VERTEX_POINT ( 'NONE', #121537 ) ;
#72559=CIRCLE ( 'NONE', #126835, 0.1000000000000000472 ) ;
#72560=DIRECTION ( 'NONE',  ( -0.000000000000000000, 1.000000000000000000, -0.000000000000000000 ) ) ;
#72561=CARTESIAN_POINT ( 'NONE',  ( -8.750000000000007105, 2.500000000000000000, 7.188010851410848723 ) ) ;
#72562=CIRCLE ( 'NONE', #65996, 0.1000000000000002554 ) ;
#72563=ORIENTED_EDGE ( 'NONE', *, *, #123010, .F. ) ;
#72565=CIRCLE ( 'NONE', #108047, 0.09999999999999982514 ) ;
#72566=CIRCLE ( 'NONE', #45376, 0.09999999999999982514 ) ;
#72567=DIRECTION ( 'NONE',  ( 0.000000000000000000, 0.000000000000000000, -1.000000000000000000 ) ) ;
#72568=LINE ( 'NONE', #22186, #24565 ) ;
#72569=ORIENTED_EDGE ( 'NONE', *, *, #23159, .T. ) ;
#72570=CARTESIAN_POINT ( 'NONE',  ( 4.399999999999939071, 2.500000000000000000, 0.2464101615137736789 ) ) ;
#72571=DIRECTION ( 'NONE',  ( 0.000000000000000000, 1.000000000000000000, 0.000000000000000000 ) ) ;
#72572=ORIENTED_EDGE ( 'NONE', *, *, #111932, .T. ) ;
#72573=VERTEX_POINT ( 'NONE', #23333 ) ;
#72574=ORIENTED_EDGE ( 'NONE', *, *, #80343, .T. ) ;
#72575=EDGE_LOOP ( 'NONE', ( #86114, #81168, #109152, #14420 ) ) ;
#72576=CARTESIAN_POINT ( 'NONE',  ( -6.071532165918824830E-15, 2.500000000000000000, -4.330127018922201643 ) ) ;
#72577=LINE ( 'NONE', #89632, #13192 ) ;
#72578=CARTESIAN_POINT ( 'NONE',  ( 21.24754738303297330, 0.7337760880902002292, -4.182111650399407132 ) ) ;
#72579=DIRECTION ( 'NONE',  ( -4.274815082592931898E-19, -0.9999939076577903929, -0.003490651415223739937 ) ) ;
#72580=ORIENTED_EDGE ( 'NONE', *, *, #105540, .T. ) ;
#72581=CARTESIAN_POINT ( 'NONE',  ( 14.14999999999989733, 12.50000000000000000, 1.472243186433545459 ) ) ;
#72583=ORIENTED_EDGE ( 'NONE', *, *, #37618, .F. ) ;
#72584=DIRECTION ( 'NONE',  ( -0.000000000000000000, -1.000000000000000000, -0.000000000000000000 ) ) ;
#72585=CARTESIAN_POINT ( 'NONE',  ( 7.306656945318285246, -1.500000000000379918, -9.704971168320719599 ) ) ;
#72586=FACE_OUTER_BOUND ( 'NONE', #22192, .T. ) ;
#72587=CARTESIAN_POINT ( 'NONE',  ( -0.2000000000000404232, 2.500000000000000000, 4.083716857408421497 ) ) ;
#72588=EDGE_CURVE ( 'NONE', #91712, #28130, #77346, .T. ) ;
#72589=ORIENTED_EDGE ( 'NONE', *, *, #49495, .T. ) ;
#72590=VECTOR ( 'NONE', #513, 1000.000000000000000 ) ;
#72591=VERTEX_POINT ( 'NONE', #71813 ) ;
#72592=ORIENTED_EDGE ( 'NONE', *, *, #123583, .T. ) ;
#72593=CARTESIAN_POINT ( 'NONE',  ( -1.450000000000035039, 2.500000000000000000, -6.741600689897077281 ) ) ;
#72594=CARTESIAN_POINT ( 'NONE',  ( -10.80000000000000071, 2.500000000000000000, -2.276824562219559311E-15 ) ) ;
#72595=EDGE_CURVE ( 'NONE', #92706, #46131, #62645, .T. ) ;
#72596=DIRECTION ( 'NONE',  ( -0.000000000000000000, -1.000000000000000000, -0.000000000000000000 ) ) ;
#72597=FACE_BOUND ( 'NONE', #27179, .T. ) ;
#72598=FACE_OUTER_BOUND ( 'NONE', #6546, .T. ) ;
#72599=PLANE ( 'NONE',  #36139 ) ;
#72600=VECTOR ( 'NONE', #44401, 1000.000000000000000 ) ;
#72601=AXIS2_PLACEMENT_3D ( 'NONE', #110752, #42029, #11911 ) ;
#72602=CARTESIAN_POINT ( 'NONE',  ( 7.299999999999926104, 12.50000000000000000, 4.676537180435972552 ) ) ;
#72604=CARTESIAN_POINT ( 'NONE',  ( 0.6499999999999566125, 2.500000000000000000, -6.841600689897077814 ) ) ;
#72605=CARTESIAN_POINT ( 'NONE',  ( 3.549999999999941203, 2.500000000000000000, 6.148780366869520897 ) ) ;
#72606=VERTEX_POINT ( 'NONE', #1762 ) ;
#72607=VECTOR ( 'NONE', #27955, 1000.000000000000000 ) ;
#72608=CIRCLE ( 'NONE', #18204, 0.1000000000000002554 ) ;
#72609=VECTOR ( 'NONE', #18524, 1000.000000000000000 ) ;
#72611=ORIENTED_EDGE ( 'NONE', *, *, #28597, .F. ) ;
#72612=ORIENTED_EDGE ( 'NONE', *, *, #121845, .F. ) ;
#72613=DIRECTION ( 'NONE',  ( -0.000000000000000000, -1.000000000000000000, -0.000000000000000000 ) ) ;
#72614=FACE_OUTER_BOUND ( 'NONE', #24807, .T. ) ;
#72615=FACE_BOUND ( 'NONE', #57596, .T. ) ;
#72616=DIRECTION ( 'NONE',  ( -4.274815082592931898E-19, -0.9999939076577903929, -0.003490651415223739937 ) ) ;
#72617=EDGE_CURVE ( 'NONE', #110704, #99929, #52170, .T. ) ;
#72618=ORIENTED_EDGE ( 'NONE', *, *, #30254, .T. ) ;
#72619=EDGE_CURVE ( 'NONE', #93363, #125180, #48100, .T. ) ;
#72620=CARTESIAN_POINT ( 'NONE',  ( -0.8500000000000395017, 12.50000000000000000, 6.495190528383297135 ) ) ;
#72621=EDGE_CURVE ( 'NONE', #76276, #105557, #98262, .T. ) ;
#72622=DIRECTION ( 'NONE',  ( 0.000000000000000000, -0.9999939076577903929, 0.003490651415223739937 ) ) ;
#72623=ADVANCED_FACE ( 'NONE', ( #122205 ), #50881, .T. ) ;
#72624=AXIS2_PLACEMENT_3D ( 'NONE', #7911, #47863, #98228 ) ;
#72626=EDGE_LOOP ( 'NONE', ( #100747, #53317, #124374, #31624 ) ) ;
#72627=DIRECTION ( 'NONE',  ( -0.000000000000000000, 1.000000000000000000, -0.000000000000000000 ) ) ;
#72628=AXIS2_PLACEMENT_3D ( 'NONE', #79659, #49820, #120474 ) ;
#72629=CARTESIAN_POINT ( 'NONE',  ( 9.799999999999918998, 12.50000000000000000, -0.3464101615137782364 ) ) ;
#72630=EDGE_CURVE ( 'NONE', #15958, #116681, #121571, .T. ) ;
#72632=DIRECTION ( 'NONE',  ( -0.000000000000000000, -1.000000000000000000, -0.000000000000000000 ) ) ;
#72633=EDGE_CURVE ( 'NONE', #81018, #89491, #75598, .T. ) ;
#72634=DIRECTION ( 'NONE',  ( 0.000000000000000000, 0.000000000000000000, 1.000000000000000000 ) ) ;
#72635=AXIS2_PLACEMENT_3D ( 'NONE', #65704, #46077, #76179 ) ;
#72636=CIRCLE ( 'NONE', #30788, 0.06509327318403745899 ) ;
#72637=ORIENTED_EDGE ( 'NONE', *, *, #94026, .F. ) ;
#72638=AXIS2_PLACEMENT_3D ( 'NONE', #15022, #125010, #103445 ) ;
#72639=CARTESIAN_POINT ( 'NONE',  ( 13.54999999999989768, 2.500000000000000000, -2.611473670974877592 ) ) ;
#72640=EDGE_CURVE ( 'NONE', #47032, #92847, #94470, .T. ) ;
#72641=DIRECTION ( 'NONE',  ( -0.000000000000000000, 1.000000000000000000, -0.000000000000000000 ) ) ;
#72642=DIRECTION ( 'NONE',  ( -0.000000000000000000, -1.000000000000000000, -0.000000000000000000 ) ) ;
#72643=ORIENTED_EDGE ( 'NONE', *, *, #111103, .T. ) ;
#72644=EDGE_LOOP ( 'NONE', ( #4138, #61998, #13340, #67727 ) ) ;
#72645=AXIS2_PLACEMENT_3D ( 'NONE', #127553, #39202, #97442 ) ;
#72646=EDGE_CURVE ( 'NONE', #10174, #119726, #125769, .T. ) ;
#72647=DIRECTION ( 'NONE',  ( 0.000000000000000000, 1.000000000000000000, 0.000000000000000000 ) ) ;
#72648=EDGE_CURVE ( 'NONE', #63986, #45554, #94020, .T. ) ;
#72650=CARTESIAN_POINT ( 'NONE',  ( 10.59999999999990905, 2.500000000000000000, -3.983716857408426293 ) ) ;
#72651=FACE_OUTER_BOUND ( 'NONE', #46615, .T. ) ;
#72652=VECTOR ( 'NONE', #53490, 1000.000000000000000 ) ;
#72653=ORIENTED_EDGE ( 'NONE', *, *, #111009, .T. ) ;
#72654=DIRECTION ( 'NONE',  ( 0.000000000000000000, 1.000000000000000000, 0.000000000000000000 ) ) ;
#72657=CARTESIAN_POINT ( 'NONE',  ( 7.049999999999928768, 12.50000000000000000, 6.495190528383297135 ) ) ;
#72658=DIRECTION ( 'NONE',  ( 0.000000000000000000, 0.000000000000000000, 1.000000000000000000 ) ) ;
#72659=EDGE_CURVE ( 'NONE', #48660, #5028, #65840, .T. ) ;
#72660=ORIENTED_EDGE ( 'NONE', *, *, #3032, .T. ) ;
#72661=ORIENTED_EDGE ( 'NONE', *, *, #105736, .F. ) ;
#72663=ORIENTED_EDGE ( 'NONE', *, *, #66259, .T. ) ;
#72664=CARTESIAN_POINT ( 'NONE',  ( -12.29999999999999361, 2.500000000000000000, 4.083716857408420609 ) ) ;
#72665=VERTEX_POINT ( 'NONE', #16721 ) ;
#72666=ORIENTED_EDGE ( 'NONE', *, *, #10504, .T. ) ;
#72668=AXIS2_PLACEMENT_3D ( 'NONE', #64729, #85010, #124304 ) ;
#72669=DIRECTION ( 'NONE',  ( 0.000000000000000000, 0.000000000000000000, -1.000000000000000000 ) ) ;
#72670=PLANE ( 'NONE',  #29729 ) ;
#72671=DIRECTION ( 'NONE',  ( 0.000000000000000000, 1.000000000000000000, 0.000000000000000000 ) ) ;
#72672=CARTESIAN_POINT ( 'NONE',  ( -10.40000000000000213, 2.500000000000000000, 0.7928203230275495672 ) ) ;
#72674=FACE_OUTER_BOUND ( 'NONE', #59277, .T. ) ;
#72675=FACE_OUTER_BOUND ( 'NONE', #6302, .T. ) ;
#72676=CARTESIAN_POINT ( 'NONE',  ( -13.09999999999999076, 12.50000000000000000, 4.048810130592458201 ) ) ;
#72677=DIRECTION ( 'NONE',  ( 0.000000000000000000, 0.000000000000000000, -1.000000000000000000 ) ) ;
#72678=AXIS2_PLACEMENT_3D ( 'NONE', #114344, #24687, #104527 ) ;
#72679=ORIENTED_EDGE ( 'NONE', *, *, #41155, .F. ) ;
#72680=ADVANCED_FACE ( 'NONE', ( #95317 ), #77744, .T. ) ;
#72681=AXIS2_PLACEMENT_3D ( 'NONE', #102354, #12655, #112815 ) ;
#72682=EDGE_CURVE ( 'NONE', #85724, #58412, #65129, .T. ) ;
#72683=CARTESIAN_POINT ( 'NONE',  ( 15.39999999999989022, 2.500000000000000000, -0.1000000000000023925 ) ) ;
#72684=ORIENTED_EDGE ( 'NONE', *, *, #86705, .T. ) ;
#72685=ORIENTED_EDGE ( 'NONE', *, *, #39372, .F. ) ;
#72686=FACE_OUTER_BOUND ( 'NONE', #100888, .T. ) ;
#72687=DIRECTION ( 'NONE',  ( 0.000000000000000000, 0.000000000000000000, -1.000000000000000000 ) ) ;
#72688=DIRECTION ( 'NONE',  ( -4.274815082592931898E-19, -0.9999939076577903929, -0.003490651415223739937 ) ) ;
#72689=AXIS2_PLACEMENT_3D ( 'NONE', #76227, #97145, #55926 ) ;
#72690=DIRECTION ( 'NONE',  ( -0.000000000000000000, 1.000000000000000000, -0.000000000000000000 ) ) ;
#72692=AXIS2_PLACEMENT_3D ( 'NONE', #39916, #97522, #50363 ) ;
#72693=CARTESIAN_POINT ( 'NONE',  ( -14.34999999999998543, 12.50000000000000000, 2.511473670974877503 ) ) ;
#72694=DIRECTION ( 'NONE',  ( 0.000000000000000000, 0.000000000000000000, 1.000000000000000000 ) ) ;
#72695=DIRECTION ( 'NONE',  ( 0.000000000000000000, -0.000000000000000000, 1.000000000000000000 ) ) ;
#72696=ORIENTED_EDGE ( 'NONE', *, *, #123890, .F. ) ;
#72697=ORIENTED_EDGE ( 'NONE', *, *, #124484, .F. ) ;
#72698=CONICAL_SURFACE ( 'NONE', #83170, 0.09999999999999982514, 0.003490658503988666988 ) ;
#72699=VERTEX_POINT ( 'NONE', #65183 ) ;
#72700=EDGE_LOOP ( 'NONE', ( #63074, #4294 ) ) ;
#72701=AXIS2_PLACEMENT_3D ( 'NONE', #108273, #127916, #27142 ) ;
#72702=ORIENTED_EDGE ( 'NONE', *, *, #31938, .F. ) ;
#72703=DIRECTION ( 'NONE',  ( 0.000000000000000000, 0.000000000000000000, -1.000000000000000000 ) ) ;
#72704=CARTESIAN_POINT ( 'NONE',  ( 7.899999999999921307, 2.500000000000000000, 0.09999999999999761857 ) ) ;
#72705=CONICAL_SURFACE ( 'NONE', #116607, 0.1000000000000002554, 0.003490658503988666988 ) ;
#72706=DIRECTION ( 'NONE',  ( -4.274815082592931898E-19, -0.9999939076577903929, -0.003490651415223739937 ) ) ;
#72707=DIRECTION ( 'NONE',  ( 0.000000000000000000, 0.000000000000000000, 1.000000000000000000 ) ) ;
#72708=CARTESIAN_POINT ( 'NONE',  ( 3.749999999999976907, 12.50000000000000000, 2.165063509461097713 ) ) ;
#72709=EDGE_LOOP ( 'NONE', ( #60876, #35928, #75306, #84725 ) ) ;
#72710=CARTESIAN_POINT ( 'NONE',  ( 7.499999999999925393, 2.500000000000000000, -0.7928203230275542301 ) ) ;
#72711=DIRECTION ( 'NONE',  ( 0.000000000000000000, -0.000000000000000000, 1.000000000000000000 ) ) ;
#72712=DIRECTION ( 'NONE',  ( 0.000000000000000000, 1.000000000000000000, 0.000000000000000000 ) ) ;
#72713=CIRCLE ( 'NONE', #16244, 0.1000000000000000472 ) ;
#72714=CONICAL_SURFACE ( 'NONE', #112432, 0.1000000000000002554, 0.003490658503988666988 ) ;
#72715=CARTESIAN_POINT ( 'NONE',  ( 0.1999999999999562961, 12.50000000000000000, 4.676537180435972552 ) ) ;
#72716=EDGE_CURVE ( 'NONE', #63975, #62965, #48423, .T. ) ;
#72717=ORIENTED_EDGE ( 'NONE', *, *, #51746, .T. ) ;
#72718=CIRCLE ( 'NONE', #53934, 0.09999999999999982514 ) ;
#72719=ORIENTED_EDGE ( 'NONE', *, *, #28759, .T. ) ;
#72720=ORIENTED_EDGE ( 'NONE', *, *, #58700, .F. ) ;
#72721=DIRECTION ( 'NONE',  ( 0.000000000000000000, 0.000000000000000000, 1.000000000000000000 ) ) ;
#72722=AXIS2_PLACEMENT_3D ( 'NONE', #10626, #49963, #29655 ) ;
#72723=CIRCLE ( 'NONE', #16254, 0.09999999999999982514 ) ;
#72724=CARTESIAN_POINT ( 'NONE',  ( -4.800000000000028244, 2.500000000000000000, -3.883716857408426648 ) ) ;
#72725=FACE_OUTER_BOUND ( 'NONE', #1068, .T. ) ;
#72727=VECTOR ( 'NONE', #65973, 1000.000000000000000 ) ;
#72728=ADVANCED_FACE ( 'NONE', ( #85492 ), #33845, .T. ) ;
#72729=EDGE_LOOP ( 'NONE', ( #103227, #78601 ) ) ;
#72730=CARTESIAN_POINT ( 'NONE',  ( -7.300000000000016698, 2.500000000000000000, -0.2464101615137783419 ) ) ;
#72731=DIRECTION ( 'NONE',  ( 0.000000000000000000, 0.000000000000000000, 1.000000000000000000 ) ) ;
#72732=CIRCLE ( 'NONE', #14126, 0.06509327318403745899 ) ;
#72733=DIRECTION ( 'NONE',  ( 0.000000000000000000, 0.000000000000000000, 1.000000000000000000 ) ) ;
#72734=EDGE_CURVE ( 'NONE', #91134, #54383, #2435, .T. ) ;
#72735=DIRECTION ( 'NONE',  ( 0.000000000000000000, 0.000000000000000000, 1.000000000000000000 ) ) ;
#72736=AXIS2_PLACEMENT_3D ( 'NONE', #53845, #123236, #73469 ) ;
#72737=AXIS2_PLACEMENT_3D ( 'NONE', #76764, #96381, #26381 ) ;
#72738=DIRECTION ( 'NONE',  ( 0.000000000000000000, 0.000000000000000000, 1.000000000000000000 ) ) ;
#72739=EDGE_LOOP ( 'NONE', ( #104484, #39839 ) ) ;
#72741=VERTEX_POINT ( 'NONE', #125417 ) ;
#72742=EDGE_CURVE ( 'NONE', #41595, #93259, #42166, .T. ) ;
#72743=CARTESIAN_POINT ( 'NONE',  ( 11.24999999999994493, 12.50000000000000000, -2.230156782645139391 ) ) ;
#72744=CARTESIAN_POINT ( 'NONE',  ( -6.650000000000015454, 2.500000000000000000, 2.857883832488649301 ) ) ;
#72745=CARTESIAN_POINT ( 'NONE',  ( -9.150000000000009237, 12.50000000000000000, -1.537336459617587581 ) ) ;
#72746=CARTESIAN_POINT ( 'NONE',  ( -3.750000000000027978, 12.50000000000000000, 7.253104124594885960 ) ) ;
#72747=VERTEX_POINT ( 'NONE', #106416 ) ;
#72748=ORIENTED_EDGE ( 'NONE', *, *, #87845, .T. ) ;
#72749=DIRECTION ( 'NONE',  ( -0.000000000000000000, 1.000000000000000000, -0.000000000000000000 ) ) ;
#72750=LINE ( 'NONE', #102833, #55167 ) ;
#72751=CARTESIAN_POINT ( 'NONE',  ( 6.699999999999930012, 12.50000000000000000, 4.395220292106234439 ) ) ;
#72752=DIRECTION ( 'NONE',  ( 0.000000000000000000, 1.000000000000000000, 0.000000000000000000 ) ) ;
#72753=ORIENTED_EDGE ( 'NONE', *, *, #81135, .T. ) ;
#72754=CARTESIAN_POINT ( 'NONE',  ( 12.69999999999990337, 2.500000000000000000, -4.776537180435978414 ) ) ;
#72755=DIRECTION ( 'NONE',  ( 0.000000000000000000, 0.000000000000000000, -1.000000000000000000 ) ) ;
#72756=ORIENTED_EDGE ( 'NONE', *, *, #18173, .F. ) ;
#72757=CIRCLE ( 'NONE', #12111, 0.1000000000000002554 ) ;
#72758=DIRECTION ( 'NONE',  ( -0.000000000000000000, 1.000000000000000000, -0.000000000000000000 ) ) ;
#72759=VERTEX_POINT ( 'NONE', #124120 ) ;
#72760=DIRECTION ( 'NONE',  ( 0.000000000000000000, 0.000000000000000000, 1.000000000000000000 ) ) ;
#72762=CONICAL_SURFACE ( 'NONE', #66405, 0.09999999999999982514, 0.003490658503988666988 ) ;
#72763=EDGE_LOOP ( 'NONE', ( #80316, #88920 ) ) ;
#72764=DIRECTION ( 'NONE',  ( -0.000000000000000000, -1.000000000000000000, -0.000000000000000000 ) ) ;
#72766=ORIENTED_EDGE ( 'NONE', *, *, #63713, .F. ) ;
#72767=EDGE_LOOP ( 'NONE', ( #60830, #70067, #79867, #61072 ) ) ;
#72768=EDGE_CURVE ( 'NONE', #378, #64066, #56809, .T. ) ;
#72771=AXIS2_PLACEMENT_3D ( 'NONE', #64692, #66619, #73871 ) ;
#72772=EDGE_CURVE ( 'NONE', #99935, #11527, #10838, .T. ) ;
#72775=VECTOR ( 'NONE', #31385, 1000.000000000000000 ) ;
#72776=DIRECTION ( 'NONE',  ( 0.000000000000000000, 0.000000000000000000, 1.000000000000000000 ) ) ;
#72777=DIRECTION ( 'NONE',  ( -4.274815082592931898E-19, -0.9999939076577903929, -0.003490651415223739937 ) ) ;
#72778=CARTESIAN_POINT ( 'NONE',  ( 3.149999999999944400, 2.500000000000000000, 1.718653347947321386 ) ) ;
#72779=ADVANCED_FACE ( 'NONE', ( #23999 ), #54765, .T. ) ;
#72780=EDGE_CURVE ( 'NONE', #97332, #85814, #25936, .T. ) ;
#72781=DIRECTION ( 'NONE',  ( 0.000000000000000000, 0.000000000000000000, 1.000000000000000000 ) ) ;
#72782=CARTESIAN_POINT ( 'NONE',  ( 13.74999999999989697, 2.500000000000000000, 2.857883832488649301 ) ) ;
#72783=EDGE_CURVE ( 'NONE', #22216, #95241, #84191, .T. ) ;
#72784=ADVANCED_FACE ( 'NONE', ( #24641 ), #64556, .T. ) ;
#72785=CIRCLE ( 'NONE', #114624, 0.1000000000000000472 ) ;
#72786=ORIENTED_EDGE ( 'NONE', *, *, #2076, .T. ) ;
#72787=ORIENTED_EDGE ( 'NONE', *, *, #31848, .T. ) ;
#72788=DIRECTION ( 'NONE',  ( 0.000000000000000000, 1.000000000000000000, 0.000000000000000000 ) ) ;
#72789=EDGE_CURVE ( 'NONE', #99291, #52298, #90262, .T. ) ;
#72790=EDGE_LOOP ( 'NONE', ( #36330, #75628, #62471, #120712 ) ) ;
#72791=DIRECTION ( 'NONE',  ( -0.000000000000000000, 1.000000000000000000, -0.000000000000000000 ) ) ;
#72792=CARTESIAN_POINT ( 'NONE',  ( -11.44999999999999751, 12.50000000000000000, -2.511473670974873951 ) ) ;
#72793=AXIS2_PLACEMENT_3D ( 'NONE', #44698, #115335, #116002 ) ;
#72794=CARTESIAN_POINT ( 'NONE',  ( 5.649999999999934630, 2.500000000000000000, 6.148780366869520897 ) ) ;
#72795=VERTEX_POINT ( 'NONE', #108975 ) ;
#72796=ORIENTED_EDGE ( 'NONE', *, *, #24449, .F. ) ;
#72797=FACE_BOUND ( 'NONE', #10894, .T. ) ;
#72798=VERTEX_POINT ( 'NONE', #89366 ) ;
#72799=CARTESIAN_POINT ( 'NONE',  ( -9.200000000000006395, 2.500000000000000000, 0.09999999999999761857 ) ) ;
#72800=CARTESIAN_POINT ( 'NONE',  ( 21.23528140090950345, -2.699413673072312392, 2.293764360948889802 ) ) ;
#72801=EDGE_CURVE ( 'NONE', #118526, #14213, #57325, .T. ) ;
#72802=CARTESIAN_POINT ( 'NONE',  ( 1.249999999999988454, 2.500000000000000000, -2.165063509461101710 ) ) ;
#72803=VECTOR ( 'NONE', #77202, 1000.000000000000000 ) ;
#72804=DIRECTION ( 'NONE',  ( -0.000000000000000000, -1.000000000000000000, -0.000000000000000000 ) ) ;
#72805=DIRECTION ( 'NONE',  ( 0.000000000000000000, 0.000000000000000000, -1.000000000000000000 ) ) ;
#72806=FACE_OUTER_BOUND ( 'NONE', #19918, .T. ) ;
#72807=CARTESIAN_POINT ( 'NONE',  ( 1.849999999999949685, 2.500000000000000000, 1.718653347947321386 ) ) ;
#72809=PLANE ( 'NONE',  #53742 ) ;
#72810=CARTESIAN_POINT ( 'NONE',  ( 11.44999999999990692, 2.500000000000000000, -6.741600689897078169 ) ) ;
#72811=AXIS2_PLACEMENT_3D ( 'NONE', #18565, #106300, #127870 ) ;
#72812=AXIS2_PLACEMENT_3D ( 'NONE', #75234, #74595, #126279 ) ;
#72813=DIRECTION ( 'NONE',  ( -0.000000000000000000, 1.000000000000000000, -0.000000000000000000 ) ) ;
#72814=ORIENTED_EDGE ( 'NONE', *, *, #29296, .F. ) ;
#72815=AXIS2_PLACEMENT_3D ( 'NONE', #42653, #90416, #52440 ) ;
#72816=ORIENTED_EDGE ( 'NONE', *, *, #33937, .F. ) ;
#72817=ORIENTED_EDGE ( 'NONE', *, *, #2875, .T. ) ;
#72818=DIRECTION ( 'NONE',  ( -0.000000000000000000, -1.000000000000000000, -0.000000000000000000 ) ) ;
#72819=VERTEX_POINT ( 'NONE', #118170 ) ;
#72820=FACE_OUTER_BOUND ( 'NONE', #122465, .T. ) ;
#72821=VERTEX_POINT ( 'NONE', #128674 ) ;
#72822=ORIENTED_EDGE ( 'NONE', *, *, #35216, .T. ) ;
#72823=VERTEX_POINT ( 'NONE', #126714 ) ;
#72824=DIRECTION ( 'NONE',  ( 0.000000000000000000, 0.000000000000000000, 1.000000000000000000 ) ) ;
#72825=CARTESIAN_POINT ( 'NONE',  ( 3.099999999999945466, 12.50000000000000000, -3.918623584224389056 ) ) ;
#72826=DIRECTION ( 'NONE',  ( 0.000000000000000000, 0.000000000000000000, -1.000000000000000000 ) ) ;
#72827=DIRECTION ( 'NONE',  ( 0.000000000000000000, 1.000000000000000000, 0.000000000000000000 ) ) ;
#72828=FACE_OUTER_BOUND ( 'NONE', #52271, .T. ) ;
#72829=CONICAL_SURFACE ( 'NONE', #68603, 0.09999999999999982514, 0.003490658503988666988 ) ;
#72830=VERTEX_POINT ( 'NONE', #76963 ) ;
#72831=DIRECTION ( 'NONE',  ( -0.000000000000000000, -1.000000000000000000, -0.000000000000000000 ) ) ;
#72832=ORIENTED_EDGE ( 'NONE', *, *, #129092, .F. ) ;
#72833=CIRCLE ( 'NONE', #7970, 0.1000000000000000472 ) ;
#72834=AXIS2_PLACEMENT_3D ( 'NONE', #108782, #39443, #115 ) ;
#72835=ORIENTED_EDGE ( 'NONE', *, *, #55612, .T. ) ;
#72836=EDGE_CURVE ( 'NONE', #84933, #120640, #48153, .T. ) ;
#72838=LINE ( 'NONE', #30353, #65169 ) ;
#72839=ORIENTED_EDGE ( 'NONE', *, *, #63030, .F. ) ;
#72840=VERTEX_POINT ( 'NONE', #127994 ) ;
#72841=ORIENTED_EDGE ( 'NONE', *, *, #65368, .F. ) ;
#72842=EDGE_CURVE ( 'NONE', #109254, #127530, #17374, .T. ) ;
#72843=CARTESIAN_POINT ( 'NONE',  ( 10.39999999999990976, 2.500000000000000000, 4.330127018922196314 ) ) ;
#72844=CARTESIAN_POINT ( 'NONE',  ( 4.399999999999937295, 12.50000000000000000, 4.676537180435972552 ) ) ;
#72845=CARTESIAN_POINT ( 'NONE',  ( -5.450000000000019718, 2.500000000000000000, 2.065063509461097624 ) ) ;
#72846=CARTESIAN_POINT ( 'NONE',  ( -8.749999999999975131, 2.500000000000000000, 2.165063509461097713 ) ) ;
#72847=VECTOR ( 'NONE', #72622, 1000.000000000000000 ) ;
#72848=CARTESIAN_POINT ( 'NONE',  ( 3.549999999999942091, 12.50000000000000000, 2.511473670974873507 ) ) ;
#72849=EDGE_LOOP ( 'NONE', ( #121210, #30687 ) ) ;
#72850=AXIS2_PLACEMENT_3D ( 'NONE', #23609, #13124, #93009 ) ;
#72851=CARTESIAN_POINT ( 'NONE',  ( -2.500000000000031086, 2.500000000000000000, 3.737306695894644371 ) ) ;
#72852=AXIS2_PLACEMENT_3D ( 'NONE', #87956, #117410, #76879 ) ;
#72853=ORIENTED_EDGE ( 'NONE', *, *, #9069, .T. ) ;
#72855=AXIS2_PLACEMENT_3D ( 'NONE', #54160, #76378, #24699 ) ;
#72856=ORIENTED_EDGE ( 'NONE', *, *, #88298, .T. ) ;
#72857=DIRECTION ( 'NONE',  ( -0.000000000000000000, -1.000000000000000000, -0.000000000000000000 ) ) ;
#72858=VERTEX_POINT ( 'NONE', #107712 ) ;
#72859=VECTOR ( 'NONE', #42233, 1000.000000000000000 ) ;
#72861=CIRCLE ( 'NONE', #62409, 0.1000000000000000472 ) ;
#72862=VECTOR ( 'NONE', #64189, 1000.000000000000000 ) ;
#72863=CARTESIAN_POINT ( 'NONE',  ( -1.650000000000034328, 2.500000000000000000, -2.265063509461101798 ) ) ;
#72864=ORIENTED_EDGE ( 'NONE', *, *, #125426, .T. ) ;
#72865=EDGE_LOOP ( 'NONE', ( #41957, #118660, #48325, #58623 ) ) ;
#72866=CARTESIAN_POINT ( 'NONE',  ( -4.999999999999986677, 2.500000000000000000, 4.430127018922196847 ) ) ;
#72867=CARTESIAN_POINT ( 'NONE',  ( 11.44999999999990870, 2.500000000000000000, 6.841600689897072485 ) ) ;
#72868=CARTESIAN_POINT ( 'NONE',  ( 6.449999999999930012, 2.500000000000000000, 6.841600689897072485 ) ) ;
#72869=LINE ( 'NONE', #80765, #22157 ) ;
#72870=CIRCLE ( 'NONE', #87517, 0.09999999999999982514 ) ;
#72871=DIRECTION ( 'NONE',  ( 0.000000000000000000, 0.000000000000000000, 1.000000000000000000 ) ) ;
#72872=ADVANCED_FACE ( 'NONE', ( #97241 ), #9513, .T. ) ;
#72873=ORIENTED_EDGE ( 'NONE', *, *, #19730, .F. ) ;
#72874=CARTESIAN_POINT ( 'NONE',  ( 2.500000000000001776, -2.021986658763282207, 9.892226903609813604 ) ) ;
#72875=VERTEX_POINT ( 'NONE', #37047 ) ;
#72876=DIRECTION ( 'NONE',  ( 0.000000000000000000, -0.000000000000000000, 1.000000000000000000 ) ) ;
#72877=DIRECTION ( 'NONE',  ( -0.000000000000000000, -1.000000000000000000, -0.000000000000000000 ) ) ;
#72878=VECTOR ( 'NONE', #50918, 1000.000000000000000 ) ;
#72879=EDGE_CURVE ( 'NONE', #53654, #66522, #71498, .T. ) ;
#72880=VECTOR ( 'NONE', #39504, 1000.000000000000000 ) ;
#72881=AXIS2_PLACEMENT_3D ( 'NONE', #44366, #71398, #4413 ) ;
#72882=EDGE_CURVE ( 'NONE', #126113, #78182, #63090, .T. ) ;
#72883=ADVANCED_FACE ( 'NONE', ( #118818 ), #69337, .T. ) ;
#72885=DIRECTION ( 'NONE',  ( 0.000000000000000000, -0.000000000000000000, 1.000000000000000000 ) ) ;
#72886=DIRECTION ( 'NONE',  ( -4.274815082592931898E-19, -0.9999939076577903929, -0.003490651415223739937 ) ) ;
#72887=DIRECTION ( 'NONE',  ( 0.000000000000000000, 0.000000000000000000, -1.000000000000000000 ) ) ;
#72888=ADVANCED_FACE ( 'NONE', ( #39646 ), #88105, .T. ) ;
#72889=DIRECTION ( 'NONE',  ( 0.000000000000000000, 0.000000000000000000, 1.000000000000000000 ) ) ;
#72890=VERTEX_POINT ( 'NONE', #8209 ) ;
#72891=VECTOR ( 'NONE', #123550, 1000.000000000000000 ) ;
#72892=DIRECTION ( 'NONE',  ( 0.000000000000000000, 0.000000000000000000, 1.000000000000000000 ) ) ;
#72893=CARTESIAN_POINT ( 'NONE',  ( -3.350000000000032507, 2.500000000000000000, -6.395190528383301931 ) ) ;
#72894=FACE_OUTER_BOUND ( 'NONE', #50742, .T. ) ;
#72895=EDGE_CURVE ( 'NONE', #100735, #106700, #44308, .T. ) ;
#72896=VERTEX_POINT ( 'NONE', #29169 ) ;
#72897=EDGE_CURVE ( 'NONE', #37017, #97094, #31805, .T. ) ;
#72898=CIRCLE ( 'NONE', #118954, 0.06509327318403745899 ) ;
#72899=CARTESIAN_POINT ( 'NONE',  ( -15.19999999999998330, 12.50000000000000000, 0.3464101615137758494 ) ) ;
#72900=CIRCLE ( 'NONE', #70837, 0.1000000000000000472 ) ;
#72901=EDGE_LOOP ( 'NONE', ( #11745, #21854, #90088, #38225 ) ) ;
#72902=ORIENTED_EDGE ( 'NONE', *, *, #120891, .F. ) ;
#72903=CARTESIAN_POINT ( 'NONE',  ( -9.350000000000006750, 2.500000000000000000, 1.918653347947321564 ) ) ;
#72904=VERTEX_POINT ( 'NONE', #49459 ) ;
#72905=CARTESIAN_POINT ( 'NONE',  ( 16.53754090006383848, -0.4856821978172663479, -6.114873053049103113 ) ) ;
#72906=CARTESIAN_POINT ( 'NONE',  ( 0.8499999999999536815, 2.500000000000000000, 6.495190528383297135 ) ) ;
#72907=DIRECTION ( 'NONE',  ( 0.000000000000000000, 0.000000000000000000, -1.000000000000000000 ) ) ;
#72908=EDGE_LOOP ( 'NONE', ( #35578, #93674 ) ) ;
#72909=CARTESIAN_POINT ( 'NONE',  ( -9.350000000000006750, 12.50000000000000000, 1.818653347947321475 ) ) ;
#72910=CIRCLE ( 'NONE', #118964, 0.06509327318403745899 ) ;
#72911=VECTOR ( 'NONE', #12999, 1000.000000000000000 ) ;
#72912=DIRECTION ( 'NONE',  ( 0.000000000000000000, 0.000000000000000000, 1.000000000000000000 ) ) ;
#72913=AXIS2_PLACEMENT_3D ( 'NONE', #125421, #53472, #55395 ) ;
#72914=ORIENTED_EDGE ( 'NONE', *, *, #20282, .F. ) ;
#72915=AXIS2_PLACEMENT_3D ( 'NONE', #91528, #20851, #1206 ) ;
#72916=ORIENTED_EDGE ( 'NONE', *, *, #42899, .F. ) ;
#72917=ORIENTED_EDGE ( 'NONE', *, *, #76130, .F. ) ;
#72918=DIRECTION ( 'NONE',  ( 0.000000000000000000, 0.000000000000000000, 1.000000000000000000 ) ) ;
#72919=DIRECTION ( 'NONE',  ( 0.000000000000000000, -0.000000000000000000, 1.000000000000000000 ) ) ;
#72920=DIRECTION ( 'NONE',  ( -0.000000000000000000, -1.000000000000000000, -0.000000000000000000 ) ) ;
#72921=ORIENTED_EDGE ( 'NONE', *, *, #60258, .F. ) ;
#72922=DIRECTION ( 'NONE',  ( 0.000000000000000000, 1.000000000000000000, 0.000000000000000000 ) ) ;
#72923=CARTESIAN_POINT ( 'NONE',  ( 6.449999999999931788, 2.500000000000000000, -2.511473670974877948 ) ) ;
#72924=ORIENTED_EDGE ( 'NONE', *, *, #19368, .T. ) ;
#72925=DIRECTION ( 'NONE',  ( 0.000000000000000000, 1.000000000000000000, 0.000000000000000000 ) ) ;
#72926=DIRECTION ( 'NONE',  ( 0.000000000000000000, -0.000000000000000000, 1.000000000000000000 ) ) ;
#72928=ADVANCED_FACE ( 'NONE', ( #18029 ), #81860, .T. ) ;
#72929=CARTESIAN_POINT ( 'NONE',  ( 3.749999999999942268, 2.500000000000000000, 1.472243186433545459 ) ) ;
#72932=EDGE_CURVE ( 'NONE', #58787, #90838, #27860, .T. ) ;
#72933=CARTESIAN_POINT ( 'NONE',  ( -8.350000000000013856, 12.50000000000000000, -5.737276932171707422 ) ) ;
#72934=LINE ( 'NONE', #23179, #8565 ) ;
#72935=ADVANCED_FACE ( 'NONE', ( #119448 ), #29797, .T. ) ;
#72936=ADVANCED_FACE ( 'NONE', ( #107051 ), #13996, .T. ) ;
#72937=CIRCLE ( 'NONE', #45753, 0.09999999999999982514 ) ;
#72938=VECTOR ( 'NONE', #96182, 1000.000000000000000 ) ;
#72939=ORIENTED_EDGE ( 'NONE', *, *, #6399, .T. ) ;
#72940=EDGE_LOOP ( 'NONE', ( #105577, #18082, #59233, #3980 ) ) ;
#72941=EDGE_CURVE ( 'NONE', #129288, #27568, #50103, .T. ) ;
#72942=ORIENTED_EDGE ( 'NONE', *, *, #101211, .T. ) ;
#72943=EDGE_LOOP ( 'NONE', ( #30898, #31343 ) ) ;
#72944=CARTESIAN_POINT ( 'NONE',  ( 0.5999999999999612310, 12.50000000000000000, -0.2813168883297386680 ) ) ;
#72945=CARTESIAN_POINT ( 'NONE',  ( 9.999999999999952038, 2.500000000000000000, -2.276824562219559311E-15 ) ) ;
#72947=VERTEX_POINT ( 'NONE', #120114 ) ;
#72948=FACE_BOUND ( 'NONE', #118074, .T. ) ;
#72949=FACE_OUTER_BOUND ( 'NONE', #20726, .T. ) ;
#72950=CARTESIAN_POINT ( 'NONE',  ( 3.749999999999976907, 12.50000000000000000, 2.099970236277060032 ) ) ;
#72951=AXIS2_PLACEMENT_3D ( 'NONE', #70297, #29718, #48730 ) ;
#72952=AXIS2_PLACEMENT_3D ( 'NONE', #20843, #32627, #9732 ) ;
#72953=ADVANCED_FACE ( 'NONE', ( #122684 ), #61191, .T. ) ;
#72954=CARTESIAN_POINT ( 'NONE',  ( 1.049999999999952083, 2.500000000000000000, 6.841600689897072485 ) ) ;
#72955=CIRCLE ( 'NONE', #123125, 0.06509327318403745899 ) ;
#72956=EDGE_CURVE ( 'NONE', #109646, #98794, #34967, .T. ) ;
#72957=DIRECTION ( 'NONE',  ( 0.000000000000000000, 1.000000000000000000, 0.000000000000000000 ) ) ;
#72958=LINE ( 'NONE', #32416, #30469 ) ;
#72959=DIRECTION ( 'NONE',  ( -0.000000000000000000, 1.000000000000000000, -0.000000000000000000 ) ) ;
#72960=CARTESIAN_POINT ( 'NONE',  ( -11.04999999999999893, 12.50000000000000000, 1.818653347947321475 ) ) ;
#72961=CARTESIAN_POINT ( 'NONE',  ( -15.19999999999998153, 2.500000000000000000, -0.2464101615137759549 ) ) ;
#72963=ORIENTED_EDGE ( 'NONE', *, *, #6556, .F. ) ;
#72964=AXIS2_PLACEMENT_3D ( 'NONE', #64656, #97817, #24095 ) ;
#72965=EDGE_LOOP ( 'NONE', ( #110266, #8648 ) ) ;
#72966=EDGE_LOOP ( 'NONE', ( #3208, #49539, #82018, #100304 ) ) ;
#72967=ORIENTED_EDGE ( 'NONE', *, *, #23869, .T. ) ;
#72968=ORIENTED_EDGE ( 'NONE', *, *, #29847, .F. ) ;
#72969=ORIENTED_EDGE ( 'NONE', *, *, #51175, .F. ) ;
#72970=DIRECTION ( 'NONE',  ( 0.000000000000000000, 1.000000000000000000, 0.000000000000000000 ) ) ;
#72971=EDGE_LOOP ( 'NONE', ( #64507, #560 ) ) ;
#72972=VERTEX_POINT ( 'NONE', #121390 ) ;
#72973=AXIS2_PLACEMENT_3D ( 'NONE', #59575, #49740, #129598 ) ;
#72974=DIRECTION ( 'NONE',  ( 0.000000000000000000, 0.000000000000000000, -1.000000000000000000 ) ) ;
#72975=DIRECTION ( 'NONE',  ( -1.000000000000000000, -0.000000000000000000, -0.000000000000000000 ) ) ;
#72976=CARTESIAN_POINT ( 'NONE',  ( -3.100000000000028511, 2.500000000000000000, 0.2464101615137736789 ) ) ;
#72977=CIRCLE ( 'NONE', #43752, 0.09999999999999982514 ) ;
#72978=VERTEX_POINT ( 'NONE', #101763 ) ;
#72979=DIRECTION ( 'NONE',  ( 0.000000000000000000, 0.000000000000000000, 1.000000000000000000 ) ) ;
#72980=ORIENTED_EDGE ( 'NONE', *, *, #41005, .F. ) ;
#72981=ORIENTED_EDGE ( 'NONE', *, *, #55506, .T. ) ;
#72982=CIRCLE ( 'NONE', #95961, 0.1000000000000002554 ) ;
#72983=CARTESIAN_POINT ( 'NONE',  ( -7.700000000000014388, 2.500000000000000000, -0.2464101615137782308 ) ) ;
#72984=CARTESIAN_POINT ( 'NONE',  ( -5.650000000000023448, 12.50000000000000000, -1.818653347947326138 ) ) ;
#72985=VERTEX_POINT ( 'NONE', #72944 ) ;
#72986=AXIS2_PLACEMENT_3D ( 'NONE', #36796, #25662, #126459 ) ;
#72987=UNCERTAINTY_MEASURE_WITH_UNIT (LENGTH_MEASURE( 1.000000000000000082E-05 ), #16004, 'distance_accuracy_value', 'NONE');
#72988=EDGE_LOOP ( 'NONE', ( #104804, #38381 ) ) ;
#72989=CARTESIAN_POINT ( 'NONE',  ( 11.89999999999990443, 2.500000000000000000, 0.3464101615137736845 ) ) ;
#72990=CIRCLE ( 'NONE', #89159, 0.09999999999999982514 ) ;
#72991=EDGE_CURVE ( 'NONE', #16954, #51911, #87165, .T. ) ;
#72992=CARTESIAN_POINT ( 'NONE',  ( -4.350000000000023626, 2.500000000000000000, 2.511473670974873507 ) ) ;
#72994=LINE ( 'NONE', #91340, #37769 ) ;
#72995=DIRECTION ( 'NONE',  ( 0.000000000000000000, -0.9999939076577903929, 0.003490651415223739937 ) ) ;
#72996=CIRCLE ( 'NONE', #24880, 0.06509327318403745899 ) ;
#72997=ORIENTED_EDGE ( 'NONE', *, *, #20746, .F. ) ;
#72998=CARTESIAN_POINT ( 'NONE',  ( 14.18215599311760755, -2.499999999999999112, 6.639800458426547536 ) ) ;
#72999=ORIENTED_EDGE ( 'NONE', *, *, #61610, .F. ) ;
#73000=CARTESIAN_POINT ( 'NONE',  ( 1.449999999999952216, 2.500000000000000000, 1.818653347947321475 ) ) ;
#73001=AXIS2_PLACEMENT_3D ( 'NONE', #29891, #92028, #91382 ) ;
#73002=AXIS2_PLACEMENT_3D ( 'NONE', #13655, #14919, #112528 ) ;
#73003=ORIENTED_EDGE ( 'NONE', *, *, #85771, .T. ) ;
#73004=CARTESIAN_POINT ( 'NONE',  ( 6.449999999999928235, 12.50000000000000000, 2.576566944158910744 ) ) ;
#73005=CARTESIAN_POINT ( 'NONE',  ( -8.950000000000011724, 2.500000000000000000, -6.248780366869521430 ) ) ;
#73006=CONICAL_SURFACE ( 'NONE', #106450, 0.1000000000000002554, 0.003490658503988666988 ) ;
#73007=DIRECTION ( 'NONE',  ( 0.000000000000000000, -0.9999939076577903929, 0.003490651415223739937 ) ) ;
#73008=CARTESIAN_POINT ( 'NONE',  ( -5.800000000000022027, 2.500000000000000000, -4.430127018922202176 ) ) ;
#73009=ORIENTED_EDGE ( 'NONE', *, *, #81802, .T. ) ;
#73011=AXIS2_PLACEMENT_3D ( 'NONE', #126789, #107787, #17452 ) ;
#73012=CIRCLE ( 'NONE', #47892, 0.06509327318403745899 ) ;
#73013=CARTESIAN_POINT ( 'NONE',  ( -14.99999999999998224, 12.50000000000000000, -0.6928203230275519209 ) ) ;
#73014=ORIENTED_EDGE ( 'NONE', *, *, #69191, .F. ) ;
#73016=EDGE_LOOP ( 'NONE', ( #68597, #79584, #66065, #14461 ) ) ;
#73017=LINE ( 'NONE', #71081, #14377 ) ;
#73018=CARTESIAN_POINT ( 'NONE',  ( -1.050000000000038236, 12.50000000000000000, -1.818653347947326138 ) ) ;
#73020=LINE ( 'NONE', #32484, #13523 ) ;
#73021=CARTESIAN_POINT ( 'NONE',  ( -11.84999999999999609, 2.500000000000000000, 6.148780366869520897 ) ) ;
#73022=DIRECTION ( 'NONE',  ( -0.000000000000000000, -1.000000000000000000, -0.000000000000000000 ) ) ;
#73023=CARTESIAN_POINT ( 'NONE',  ( -2.900000000000029665, 2.500000000000000000, 3.737306695894644371 ) ) ;
#73024=AXIS2_PLACEMENT_3D ( 'NONE', #45429, #16577, #125267 ) ;
#73025=DIRECTION ( 'NONE',  ( -0.000000000000000000, -1.000000000000000000, -0.000000000000000000 ) ) ;
#73026=AXIS2_PLACEMENT_3D ( 'NONE', #81103, #43126, #31360 ) ;
#73027=ADVANCED_FACE ( 'NONE', ( #20629 ), #72524, .T. ) ;
#73028=CIRCLE ( 'NONE', #79309, 0.06509327318403745899 ) ;
#73029=ORIENTED_EDGE ( 'NONE', *, *, #119334, .T. ) ;
#73030=CARTESIAN_POINT ( 'NONE',  ( -8.950000000000006395, 12.50000000000000000, 6.841600689897072485 ) ) ;
#73031=EDGE_CURVE ( 'NONE', #118702, #3798, #1610, .T. ) ;
#73032=FACE_OUTER_BOUND ( 'NONE', #70403, .T. ) ;
#73034=CARTESIAN_POINT ( 'NONE',  ( -6.850000000000013856, 12.50000000000000000, 6.841600689897072485 ) ) ;
#73035=EDGE_CURVE ( 'NONE', #73360, #125465, #33038, .T. ) ;
#73036=CIRCLE ( 'NONE', #20807, 0.1000000000000000472 ) ;
#73037=ORIENTED_EDGE ( 'NONE', *, *, #57838, .T. ) ;
#73039=DIRECTION ( 'NONE',  ( 0.000000000000000000, 0.000000000000000000, 1.000000000000000000 ) ) ;
#73040=AXIS2_PLACEMENT_3D ( 'NONE', #69424, #127707, #87771 ) ;
#73041=FACE_OUTER_BOUND ( 'NONE', #68570, .T. ) ;
#73042=CARTESIAN_POINT ( 'NONE',  ( 5.849999999999934808, 12.50000000000000000, -5.802370205355749988 ) ) ;
#73043=ORIENTED_EDGE ( 'NONE', *, *, #17935, .F. ) ;
#73044=EDGE_CURVE ( 'NONE', #1197, #82804, #82116, .T. ) ;
#73045=EDGE_CURVE ( 'NONE', #35250, #103864, #122678, .T. ) ;
#73046=ADVANCED_FACE ( 'NONE', ( #30462 ), #57941, .T. ) ;
#73047=ADVANCED_FACE ( 'NONE', ( #32404 ), #62495, .T. ) ;
#73048=ADVANCED_FACE ( 'NONE', ( #60568 ), #21922, .T. ) ;
#73049=VECTOR ( 'NONE', #123303, 1000.000000000000000 ) ;
#73050=VERTEX_POINT ( 'NONE', #112871 ) ;
#73051=DIRECTION ( 'NONE',  ( -0.000000000000000000, 1.000000000000000000, -0.000000000000000000 ) ) ;
#73052=CIRCLE ( 'NONE', #62596, 0.06509327318403745899 ) ;
#73053=VECTOR ( 'NONE', #83993, 1000.000000000000000 ) ;
#73054=VERTEX_POINT ( 'NONE', #80840 ) ;
#73055=ORIENTED_EDGE ( 'NONE', *, *, #12475, .T. ) ;
#73056=CARTESIAN_POINT ( 'NONE',  ( 12.89999999999989733, 2.500000000000000000, 0.09999999999999761857 ) ) ;
#73057=EDGE_CURVE ( 'NONE', #101366, #113477, #32819, .T. ) ;
#73058=EDGE_LOOP ( 'NONE', ( #98334, #107121, #85892, #31103 ) ) ;
#73059=CARTESIAN_POINT ( 'NONE',  ( 18.20334136264111535, 2.532871263994777244, -4.817802756299775169 ) ) ;
#73060=DIRECTION ( 'NONE',  ( 0.000000000000000000, 0.000000000000000000, 1.000000000000000000 ) ) ;
#73061=CARTESIAN_POINT ( 'NONE',  ( -14.14999999999998614, 12.50000000000000000, 2.230156782645138946 ) ) ;
#73062=VERTEX_POINT ( 'NONE', #10158 ) ;
#73063=DIRECTION ( 'NONE',  ( 0.000000000000000000, 0.000000000000000000, 1.000000000000000000 ) ) ;
#73064=CARTESIAN_POINT ( 'NONE',  ( 12.89999999999990266, 2.500000000000000000, -4.922947341949753586 ) ) ;
#73065=ORIENTED_EDGE ( 'NONE', *, *, #119327, .T. ) ;
#73066=AXIS2_PLACEMENT_3D ( 'NONE', #40137, #38882, #118685 ) ;
#73067=CARTESIAN_POINT ( 'NONE',  ( 17.50000000000000000, 2.481874158964659571, 3.264437049506136557 ) ) ;
#73068=DIRECTION ( 'NONE',  ( 0.000000000000000000, 0.000000000000000000, -1.000000000000000000 ) ) ;
#73069=ORIENTED_EDGE ( 'NONE', *, *, #43528, .T. ) ;
#73070=ORIENTED_EDGE ( 'NONE', *, *, #109900, .F. ) ;
#73071=ORIENTED_EDGE ( 'NONE', *, *, #77663, .F. ) ;
#73072=ORIENTED_EDGE ( 'NONE', *, *, #115489, .F. ) ;
#73073=DIRECTION ( 'NONE',  ( 0.000000000000000000, 1.000000000000000000, 0.000000000000000000 ) ) ;
#73074=CARTESIAN_POINT ( 'NONE',  ( 12.07106445339185363, 1.500000000000190070, 8.629160868130334450 ) ) ;
#73075=DIRECTION ( 'NONE',  ( 0.000000000000000000, -0.000000000000000000, 1.000000000000000000 ) ) ;
#73076=FACE_BOUND ( 'NONE', #79375, .T. ) ;
#73077=ORIENTED_EDGE ( 'NONE', *, *, #1295, .F. ) ;
#73079=DIRECTION ( 'NONE',  ( 0.000000000000000000, -0.9999939076577903929, 0.003490651415223739937 ) ) ;
#73080=CARTESIAN_POINT ( 'NONE',  ( -13.09999999999999076, 12.50000000000000000, 3.918623584224383727 ) ) ;
#73082=LINE ( 'NONE', #92730, #126186 ) ;
#73083=EDGE_CURVE ( 'NONE', #76681, #101262, #18205, .T. ) ;
#73084=AXIS2_PLACEMENT_3D ( 'NONE', #48037, #38217, #26460 ) ;
#73086=EDGE_CURVE ( 'NONE', #98404, #79083, #31105, .T. ) ;
#73087=B_SPLINE_CURVE_WITH_KNOTS ( 'NONE', 3,
 ( #8374, #107872, #71023, #20637 ),
 .UNSPECIFIED., .F., .F.,
 ( 4, 4 ),
 ( 0.002015733555955077569, 0.002984807578936017093 ),
 .UNSPECIFIED. ) ;
#73088=CARTESIAN_POINT ( 'NONE',  ( 11.24999999999991118, 2.500000000000000000, 5.802370205355744659 ) ) ;
#73089=EDGE_CURVE ( 'NONE', #51142, #2098, #64184, .T. ) ;
#73091=CIRCLE ( 'NONE', #116894, 0.09999999999999982514 ) ;
#73092=ORIENTED_EDGE ( 'NONE', *, *, #97552, .T. ) ;
#73093=EDGE_LOOP ( 'NONE', ( #30354, #98716, #90093, #10307 ) ) ;
#73094=ORIENTED_EDGE ( 'NONE', *, *, #812, .T. ) ;
#73095=ORIENTED_EDGE ( 'NONE', *, *, #90171, .T. ) ;
#73096=ORIENTED_EDGE ( 'NONE', *, *, #3289, .T. ) ;
#73098=AXIS2_PLACEMENT_3D ( 'NONE', #46071, #97098, #45430 ) ;
#73099=LINE ( 'NONE', #72460, #21565 ) ;
#73100=ORIENTED_EDGE ( 'NONE', *, *, #97600, .F. ) ;
#73101=EDGE_CURVE ( 'NONE', #99888, #36155, #13686, .T. ) ;
#73102=FACE_BOUND ( 'NONE', #71538, .T. ) ;
#73103=FACE_OUTER_BOUND ( 'NONE', #65514, .T. ) ;
#73104=ADVANCED_FACE ( 'NONE', ( #75502 ), #55242, .T. ) ;
#73105=CIRCLE ( 'NONE', #110658, 0.1000000000000000472 ) ;
#73106=EDGE_CURVE ( 'NONE', #34594, #2409, #73566, .T. ) ;
#73108=EDGE_LOOP ( 'NONE', ( #42553, #6524 ) ) ;
#73109=DIRECTION ( 'NONE',  ( 0.000000000000000000, 1.000000000000000000, 0.000000000000000000 ) ) ;
#73110=DIRECTION ( 'NONE',  ( 0.000000000000000000, 0.000000000000000000, 1.000000000000000000 ) ) ;
#73111=DIRECTION ( 'NONE',  ( -0.000000000000000000, 1.000000000000000000, -0.000000000000000000 ) ) ;
#73112=ORIENTED_EDGE ( 'NONE', *, *, #6715, .T. ) ;
#73113=CARTESIAN_POINT ( 'NONE',  ( -9.350000000000006750, 2.500000000000000000, -1.918653347947325782 ) ) ;
#73114=EDGE_CURVE ( 'NONE', #70171, #110675, #9814, .T. ) ;
#73115=ORIENTED_EDGE ( 'NONE', *, *, #29472, .F. ) ;
#73116=ORIENTED_EDGE ( 'NONE', *, *, #21778, .F. ) ;
#73117=VERTEX_POINT ( 'NONE', #125886 ) ;
#73118=CARTESIAN_POINT ( 'NONE',  ( 21.23528140090950345, -2.699413673072312392, 2.293764360948889802 ) ) ;
#73119=CARTESIAN_POINT ( 'NONE',  ( -12.49999999999999289, 12.50000000000000000, -5.022947341949751454 ) ) ;
#73120=CARTESIAN_POINT ( 'NONE',  ( 9.149999999999920419, 2.500000000000000000, -7.188010851410854052 ) ) ;
#73121=ORIENTED_EDGE ( 'NONE', *, *, #121573, .F. ) ;
#73122=DIRECTION ( 'NONE',  ( 0.000000000000000000, -0.9999939076577903929, 0.003490651415223739937 ) ) ;
#73123=CIRCLE ( 'NONE', #10502, 0.1000000000000002554 ) ;
#73124=CARTESIAN_POINT ( 'NONE',  ( -10.65000000000000213, 2.500000000000000000, 2.611473670974873151 ) ) ;
#73125=VECTOR ( 'NONE', #67187, 1000.000000000000000 ) ;
#73126=CARTESIAN_POINT ( 'NONE',  ( 5.399999999999933742, 2.500000000000000000, -2.385244779468109755E-15 ) ) ;
#73127=PLANE ( 'NONE',  #60115 ) ;
#73128=EDGE_LOOP ( 'NONE', ( #97559, #99775, #100428, #116281 ) ) ;
#73129=CARTESIAN_POINT ( 'NONE',  ( -3.750000000000029310, 2.500000000000000000, -7.288010851410854585 ) ) ;
#73130=ADVANCED_FACE ( 'NONE', ( #14001 ), #35603, .T. ) ;
#73131=VERTEX_POINT ( 'NONE', #114157 ) ;
#73133=VECTOR ( 'NONE', #93292, 1000.000000000000000 ) ;
#73134=VECTOR ( 'NONE', #70734, 1000.000000000000000 ) ;
#73135=EDGE_LOOP ( 'NONE', ( #7841, #12955, #119069, #3187 ) ) ;
#73136=ORIENTED_EDGE ( 'NONE', *, *, #80025, .F. ) ;
#73137=CARTESIAN_POINT ( 'NONE',  ( 10.59999999999990905, 12.50000000000000000, -4.741630453620016006 ) ) ;
#73138=DIRECTION ( 'NONE',  ( -0.000000000000000000, 1.000000000000000000, -0.000000000000000000 ) ) ;
#73139=CARTESIAN_POINT ( 'NONE',  ( 3.749999999999978684, 2.500000000000000000, -6.495190528383302464 ) ) ;
#73140=LINE ( 'NONE', #71197, #73828 ) ;
#73141=CARTESIAN_POINT ( 'NONE',  ( -10.00000000000000355, 2.500000000000000000, 3.737306695894644371 ) ) ;
#73142=CONICAL_SURFACE ( 'NONE', #16671, 0.1000000000000002554, 0.003490658503988666988 ) ;
#73143=ORIENTED_EDGE ( 'NONE', *, *, #83244, .F. ) ;
#73144=ORIENTED_EDGE ( 'NONE', *, *, #19233, .T. ) ;
#73145=CIRCLE ( 'NONE', #108731, 0.09999999999999982514 ) ;
#73146=DIRECTION ( 'NONE',  ( 0.000000000000000000, 0.000000000000000000, 1.000000000000000000 ) ) ;
#73147=CIRCLE ( 'NONE', #56411, 0.06509327318403745899 ) ;
#73148=EDGE_CURVE ( 'NONE', #103155, #15846, #68386, .T. ) ;
#73149=DIRECTION ( 'NONE',  ( -0.000000000000000000, 1.000000000000000000, -0.000000000000000000 ) ) ;
#73150=CARTESIAN_POINT ( 'NONE',  ( -15.39999999999998082, 2.500000000000000000, 0.6928203230275518099 ) ) ;
#73151=EDGE_LOOP ( 'NONE', ( #105473, #115885, #19433, #77564 ) ) ;
#73152=VERTEX_POINT ( 'NONE', #65691 ) ;
#73153=VECTOR ( 'NONE', #108699, 1000.000000000000000 ) ;
#73154=PLANE ( 'NONE',  #112566 ) ;
#73155=AXIS2_PLACEMENT_3D ( 'NONE', #86408, #75947, #106694 ) ;
#73156=EDGE_LOOP ( 'NONE', ( #24375, #30446 ) ) ;
#73157=DIRECTION ( 'NONE',  ( -0.000000000000000000, -1.000000000000000000, -0.000000000000000000 ) ) ;
#73158=CARTESIAN_POINT ( 'NONE',  ( 0.5999999999999560130, 12.50000000000000000, -3.983716857408426293 ) ) ;
#73159=CARTESIAN_POINT ( 'NONE',  ( -5.850000000000022737, 2.500000000000000000, -2.165063509461101710 ) ) ;
#73160=ORIENTED_EDGE ( 'NONE', *, *, #14807, .T. ) ;
#73161=CARTESIAN_POINT ( 'NONE',  ( 13.34999999999989662, 12.50000000000000000, -2.165063509461101710 ) ) ;
#73162=DIRECTION ( 'NONE',  ( 0.000000000000000000, 0.000000000000000000, -1.000000000000000000 ) ) ;
#73163=DIRECTION ( 'NONE',  ( -0.000000000000000000, -1.000000000000000000, -0.000000000000000000 ) ) ;
#73164=AXIS2_PLACEMENT_3D ( 'NONE', #64857, #15088, #55050 ) ;
#73165=CARTESIAN_POINT ( 'NONE',  ( -10.20000000000000639, 2.500000000000000000, -3.883716857408422207 ) ) ;
#73166=EDGE_CURVE ( 'NONE', #121191, #70149, #105629, .T. ) ;
#73167=DIRECTION ( 'NONE',  ( 0.000000000000000000, 0.000000000000000000, 1.000000000000000000 ) ) ;
#73168=EDGE_LOOP ( 'NONE', ( #118302, #106196 ) ) ;
#73169=CARTESIAN_POINT ( 'NONE',  ( 5.849999999999933920, 2.500000000000000000, 6.495190528383297135 ) ) ;
#73170=CARTESIAN_POINT ( 'NONE',  ( 24.00496409368203743, -0.9037364215739981388, 4.313973893096084034 ) ) ;
#73171=ORIENTED_EDGE ( 'NONE', *, *, #38955, .F. ) ;
#73172=EDGE_LOOP ( 'NONE', ( #112887, #73830 ) ) ;
#73175=DIRECTION ( 'NONE',  ( -0.000000000000000000, 1.000000000000000000, -0.000000000000000000 ) ) ;
#73176=CARTESIAN_POINT ( 'NONE',  ( -7.900000000000014566, 12.50000000000000000, 0.6928203230275494784 ) ) ;
#73177=DIRECTION ( 'NONE',  ( 0.000000000000000000, 1.000000000000000000, 0.000000000000000000 ) ) ;
#73178=CARTESIAN_POINT ( 'NONE',  ( 10.84999999999991260, 2.500000000000000000, -1.472243186433550122 ) ) ;
#73179=FACE_OUTER_BOUND ( 'NONE', #94522, .T. ) ;
#73180=CARTESIAN_POINT ( 'NONE',  ( -8.350000000000012079, 12.50000000000000000, 1.472243186433545459 ) ) ;
#73181=CARTESIAN_POINT ( 'NONE',  ( -1.650000000000035216, 12.50000000000000000, -5.802370205355749988 ) ) ;
#73182=AXIS2_PLACEMENT_3D ( 'NONE', #13566, #52866, #103258 ) ;
#73183=DIRECTION ( 'NONE',  ( 0.000000000000000000, 1.000000000000000000, 0.000000000000000000 ) ) ;
#73184=VERTEX_POINT ( 'NONE', #24486 ) ;
#73185=ORIENTED_EDGE ( 'NONE', *, *, #90047, .T. ) ;
#73186=EDGE_CURVE ( 'NONE', #5233, #26170, #15283, .T. ) ;
#73187=AXIS2_PLACEMENT_3D ( 'NONE', #35064, #84128, #74968 ) ;
#73188=VECTOR ( 'NONE', #33177, 1000.000000000000000 ) ;
#73189=EDGE_LOOP ( 'NONE', ( #127491, #3698 ) ) ;
#73190=VERTEX_POINT ( 'NONE', #55867 ) ;
#73191=DIRECTION ( 'NONE',  ( -0.000000000000000000, -1.000000000000000000, -0.000000000000000000 ) ) ;
#73192=CARTESIAN_POINT ( 'NONE',  ( 3.299999999999942979, 12.50000000000000000, 4.330127018922196314 ) ) ;
#73193=EDGE_CURVE ( 'NONE', #87106, #72591, #123331, .T. ) ;
#73194=AXIS2_PLACEMENT_3D ( 'NONE', #114081, #24409, #4743 ) ;
#73195=VECTOR ( 'NONE', #29449, 1000.000000000000000 ) ;
#73196=VERTEX_POINT ( 'NONE', #124620 ) ;
#73197=DIRECTION ( 'NONE',  ( 0.000000000000000000, -0.000000000000000000, 1.000000000000000000 ) ) ;
#73198=DIRECTION ( 'NONE',  ( -0.000000000000000000, 1.000000000000000000, -0.000000000000000000 ) ) ;
#73199=DIRECTION ( 'NONE',  ( 0.000000000000000000, 1.000000000000000000, 0.000000000000000000 ) ) ;
#73200=ORIENTED_EDGE ( 'NONE', *, *, #55614, .F. ) ;
#73201=EDGE_CURVE ( 'NONE', #60164, #115875, #7741, .T. ) ;
#73202=EDGE_CURVE ( 'NONE', #48878, #102426, #94499, .T. ) ;
#73203=ADVANCED_FACE ( 'NONE', ( #23851 ), #80927, .T. ) ;
#73204=DIRECTION ( 'NONE',  ( -0.000000000000000000, 1.000000000000000000, -0.000000000000000000 ) ) ;
#73205=ADVANCED_FACE ( 'NONE', ( #53948 ), #20276, .T. ) ;
#73206=DIRECTION ( 'NONE',  ( 0.000000000000000000, 0.000000000000000000, 1.000000000000000000 ) ) ;
#73207=ORIENTED_EDGE ( 'NONE', *, *, #9383, .T. ) ;
#73208=ORIENTED_EDGE ( 'NONE', *, *, #35828, .T. ) ;
#73209=EDGE_LOOP ( 'NONE', ( #29038, #83908 ) ) ;
#73210=VERTEX_POINT ( 'NONE', #14639 ) ;
#73211=CARTESIAN_POINT ( 'NONE',  ( -4.150000000000025224, 12.50000000000000000, 6.495190528383297135 ) ) ;
#73212=ADVANCED_FACE ( 'NONE', ( #44782 ), #5584, .T. ) ;
#73213=DIRECTION ( 'NONE',  ( -4.274815082592931898E-19, -0.9999939076577903929, -0.003490651415223739937 ) ) ;
#73214=DIRECTION ( 'NONE',  ( 0.000000000000000000, 1.000000000000000000, 0.000000000000000000 ) ) ;
#73215=ADVANCED_FACE ( 'NONE', ( #57815 ), #114359, .T. ) ;
#73216=DIRECTION ( 'NONE',  ( 0.000000000000000000, 1.000000000000000000, 0.000000000000000000 ) ) ;
#73217=CIRCLE ( 'NONE', #16749, 0.06509327318403745899 ) ;
#73218=EDGE_CURVE ( 'NONE', #40642, #96734, #87891, .T. ) ;
#73219=ORIENTED_EDGE ( 'NONE', *, *, #45290, .T. ) ;
#73220=CIRCLE ( 'NONE', #8355, 0.1000000000000000472 ) ;
#73221=DIRECTION ( 'NONE',  ( 0.000000000000000000, -0.000000000000000000, 1.000000000000000000 ) ) ;
#73222=VERTEX_POINT ( 'NONE', #38172 ) ;
#73223=CARTESIAN_POINT ( 'NONE',  ( -13.34999999999999076, 12.50000000000000000, 1.537336459617586915 ) ) ;
#73224=CARTESIAN_POINT ( 'NONE',  ( 8.328334241102787416, -2.499999999999999556, -8.539519493615843615 ) ) ;
#73225=FACE_OUTER_BOUND ( 'NONE', #29193, .T. ) ;
#73226=DIRECTION ( 'NONE',  ( 0.000000000000000000, 1.000000000000000000, 0.000000000000000000 ) ) ;
#73227=AXIS2_PLACEMENT_3D ( 'NONE', #105249, #45062, #73221 ) ;
#73228=VERTEX_POINT ( 'NONE', #97728 ) ;
#73229=ORIENTED_EDGE ( 'NONE', *, *, #118265, .T. ) ;
#73230=VERTEX_POINT ( 'NONE', #17875 ) ;
#73231=CARTESIAN_POINT ( 'NONE',  ( -10.40000000000000213, 2.500000000000000000, 5.022947341949748790 ) ) ;
#73232=FACE_OUTER_BOUND ( 'NONE', #48311, .T. ) ;
#73233=FACE_OUTER_BOUND ( 'NONE', #85737, .T. ) ;
#73234=FACE_BOUND ( 'NONE', #43987, .T. ) ;
#73235=CONICAL_SURFACE ( 'NONE', #29328, 0.1000000000000002554, 0.003490658503988666988 ) ;
#73236=DIRECTION ( 'NONE',  ( -0.000000000000000000, 1.000000000000000000, -0.000000000000000000 ) ) ;
#73237=CARTESIAN_POINT ( 'NONE',  ( 7.099999999999927702, 2.500000000000000000, 4.922947341949748257 ) ) ;
#73238=DIRECTION ( 'NONE',  ( -0.000000000000000000, -1.000000000000000000, -0.000000000000000000 ) ) ;
#73239=VECTOR ( 'NONE', #98147, 1000.000000000000000 ) ;
#73240=DIRECTION ( 'NONE',  ( -0.000000000000000000, 1.000000000000000000, -0.000000000000000000 ) ) ;
#73242=CARTESIAN_POINT ( 'NONE',  ( -10.60000000000000320, 2.500000000000000000, -4.083716857408422385 ) ) ;
#73243=ORIENTED_EDGE ( 'NONE', *, *, #85790, .F. ) ;
#73244=CONICAL_SURFACE ( 'NONE', #123404, 0.09999999999999982514, 0.003490658503988666988 ) ;
#73245=CARTESIAN_POINT ( 'NONE',  ( -11.44999999999999751, 2.500000000000000000, 2.511473670974873507 ) ) ;
#73246=AXIS2_PLACEMENT_3D ( 'NONE', #75974, #16381, #23657 ) ;
#73247=EDGE_LOOP ( 'NONE', ( #67608, #92526 ) ) ;
#73248=EDGE_LOOP ( 'NONE', ( #71668, #27722 ) ) ;
#73249=LINE ( 'NONE', #62797, #102943 ) ;
#73250=EDGE_CURVE ( 'NONE', #26170, #75526, #68293, .T. ) ;
#73251=FACE_BOUND ( 'NONE', #33083, .T. ) ;
#73252=DIRECTION ( 'NONE',  ( -0.000000000000000000, 1.000000000000000000, -0.000000000000000000 ) ) ;
#73253=ADVANCED_FACE ( 'NONE', ( #8054 ), #47352, .T. ) ;
#73254=EDGE_CURVE ( 'NONE', #93836, #76693, #49538, .T. ) ;
#73255=ORIENTED_EDGE ( 'NONE', *, *, #36602, .T. ) ;
#73256=CARTESIAN_POINT ( 'NONE',  ( 43.06166283081541479, 3.066941195862745495, 4.904920240844576007 ) ) ;
#73257=CARTESIAN_POINT ( 'NONE',  ( -13.94999999999998863, 2.500000000000000000, 2.611473670974877148 ) ) ;
#73258=ORIENTED_EDGE ( 'NONE', *, *, #57622, .T. ) ;
#73259=LINE ( 'NONE', #122373, #103361 ) ;
#73261=EDGE_CURVE ( 'NONE', #7920, #111617, #45337, .T. ) ;
#73262=AXIS2_PLACEMENT_3D ( 'NONE', #120167, #1031, #1664 ) ;
#73263=VERTEX_POINT ( 'NONE', #48002 ) ;
#73264=CARTESIAN_POINT ( 'NONE',  ( 12.49999999999990052, 12.50000000000000000, 0.6928203230275494784 ) ) ;
#73265=CIRCLE ( 'NONE', #16804, 0.09999999999999982514 ) ;
#73266=CARTESIAN_POINT ( 'NONE',  ( 3.949999999999941558, 2.500000000000000000, -1.818653347947326138 ) ) ;
#73267=EDGE_LOOP ( 'NONE', ( #95694, #65719 ) ) ;
#73268=CARTESIAN_POINT ( 'NONE',  ( -12.04999999999999716, 2.500000000000000000, -6.595190528383298556 ) ) ;
#73269=DIRECTION ( 'NONE',  ( 0.000000000000000000, 0.000000000000000000, -1.000000000000000000 ) ) ;
#73270=DIRECTION ( 'NONE',  ( 0.000000000000000000, 0.000000000000000000, 1.000000000000000000 ) ) ;
#73271=EDGE_LOOP ( 'NONE', ( #59755, #61207, #77145, #88313 ) ) ;
#73272=ORIENTED_EDGE ( 'NONE', *, *, #101864, .T. ) ;
#73273=CARTESIAN_POINT ( 'NONE',  ( 5.849999999999933920, 2.500000000000000000, 5.802370205355744659 ) ) ;
#73274=EDGE_CURVE ( 'NONE', #11966, #69989, #78792, .T. ) ;
#73275=ORIENTED_EDGE ( 'NONE', *, *, #47028, .F. ) ;
#73276=DIRECTION ( 'NONE',  ( 0.000000000000000000, 0.000000000000000000, -1.000000000000000000 ) ) ;
#73277=DIRECTION ( 'NONE',  ( 0.000000000000000000, 0.000000000000000000, 1.000000000000000000 ) ) ;
#73278=ORIENTED_EDGE ( 'NONE', *, *, #127278, .T. ) ;
#73279=DIRECTION ( 'NONE',  ( -0.000000000000000000, 1.000000000000000000, -0.000000000000000000 ) ) ;
#73280=LINE ( 'NONE', #63473, #79640 ) ;
#73281=CARTESIAN_POINT ( 'NONE',  ( -3.150000000000029221, 2.500000000000000000, 2.411473670974873862 ) ) ;
#73282=CARTESIAN_POINT ( 'NONE',  ( 11.84999999999990727, 12.50000000000000000, 6.841600689897072485 ) ) ;
#73283=DIRECTION ( 'NONE',  ( 0.000000000000000000, 0.000000000000000000, 1.000000000000000000 ) ) ;
#73284=ORIENTED_EDGE ( 'NONE', *, *, #104525, .F. ) ;
#73286=CARTESIAN_POINT ( 'NONE',  ( 4.599999999999936584, 2.500000000000000000, 3.637306695894644726 ) ) ;
#73287=EDGE_LOOP ( 'NONE', ( #9320, #125333, #109265, #123053 ) ) ;
#73288=EDGE_CURVE ( 'NONE', #27754, #122264, #8682, .T. ) ;
#73290=ORIENTED_EDGE ( 'NONE', *, *, #109039, .T. ) ;
#73291=ORIENTED_EDGE ( 'NONE', *, *, #35848, .T. ) ;
#73292=ORIENTED_EDGE ( 'NONE', *, *, #121472, .T. ) ;
#73293=CARTESIAN_POINT ( 'NONE',  ( 9.599999999999917932, 12.50000000000000000, -2.276824562219559311E-15 ) ) ;
#73295=CARTESIAN_POINT ( 'NONE',  ( 6.849999999999930367, 2.500000000000000000, -6.941600689897078347 ) ) ;
#73296=VECTOR ( 'NONE', #125472, 1000.000000000000000 ) ;
#73297=CARTESIAN_POINT ( 'NONE',  ( 4.549999999999939426, 2.500000000000000000, -6.495190528383302464 ) ) ;
#73298=DIRECTION ( 'NONE',  ( 0.000000000000000000, 0.000000000000000000, 1.000000000000000000 ) ) ;
#73299=CARTESIAN_POINT ( 'NONE',  ( -1.900000000000034994, 12.50000000000000000, -4.676537180435978769 ) ) ;
#73300=DIRECTION ( 'NONE',  ( 0.000000000000000000, 0.000000000000000000, 1.000000000000000000 ) ) ;
#73301=FACE_OUTER_BOUND ( 'NONE', #77830, .T. ) ;
#73302=DIRECTION ( 'NONE',  ( 0.000000000000000000, 1.000000000000000000, 0.000000000000000000 ) ) ;
#73303=EDGE_CURVE ( 'NONE', #102426, #28344, #108180, .T. ) ;
#73305=ORIENTED_EDGE ( 'NONE', *, *, #39696, .T. ) ;
#73306=DIRECTION ( 'NONE',  ( -0.000000000000000000, -1.000000000000000000, -0.000000000000000000 ) ) ;
#73307=ORIENTED_EDGE ( 'NONE', *, *, #83449, .F. ) ;
#73308=ADVANCED_FACE ( 'NONE', ( #106896 ), #64280, .T. ) ;
#73309=ORIENTED_EDGE ( 'NONE', *, *, #103474, .F. ) ;
#73310=CARTESIAN_POINT ( 'NONE',  ( -7.300000000000014921, 2.500000000000000000, 4.576537180435972019 ) ) ;
#73311=FACE_OUTER_BOUND ( 'NONE', #25631, .T. ) ;
#73312=CARTESIAN_POINT ( 'NONE',  ( 15.39999999999989022, 2.500000000000000000, -2.385244779468109755E-15 ) ) ;
#73313=AXIS2_PLACEMENT_3D ( 'NONE', #109260, #87682, #79183 ) ;
#73315=CIRCLE ( 'NONE', #115151, 0.1000000000000002554 ) ;
#73317=LINE ( 'NONE', #124371, #94641 ) ;
#73318=DIRECTION ( 'NONE',  ( 0.000000000000000000, 1.000000000000000000, 0.000000000000000000 ) ) ;
#73319=CARTESIAN_POINT ( 'NONE',  ( 6.899999999999928413, 12.50000000000000000, -4.611443907251939756 ) ) ;
#73320=ORIENTED_EDGE ( 'NONE', *, *, #94585, .F. ) ;
#73321=LINE ( 'NONE', #118724, #51708 ) ;
#73322=CIRCLE ( 'NONE', #125552, 0.1000000000000000472 ) ;
#73323=FACE_OUTER_BOUND ( 'NONE', #79313, .T. ) ;
#73324=EDGE_LOOP ( 'NONE', ( #80211, #96617, #28182, #71790 ) ) ;
#73325=EDGE_LOOP ( 'NONE', ( #71989, #15459 ) ) ;
#73326=EDGE_CURVE ( 'NONE', #105503, #41725, #67612, .T. ) ;
#73327=AXIS2_PLACEMENT_3D ( 'NONE', #36401, #76314, #6892 ) ;
#73329=VERTEX_POINT ( 'NONE', #48636 ) ;
#73330=DIRECTION ( 'NONE',  ( 0.000000000000000000, 0.000000000000000000, 1.000000000000000000 ) ) ;
#73331=FACE_OUTER_BOUND ( 'NONE', #60592, .T. ) ;
#73332=ADVANCED_FACE ( 'NONE', ( #78760 ), #70536, .T. ) ;
#73333=CARTESIAN_POINT ( 'NONE',  ( 0.4499999999999573785, 2.500000000000000000, -6.395190528383301931 ) ) ;
#73334=CARTESIAN_POINT ( 'NONE',  ( 5.199999999999933564, 2.500000000000000000, 0.3464101615137735735 ) ) ;
#73335=DIRECTION ( 'NONE',  ( -0.000000000000000000, 1.000000000000000000, -0.000000000000000000 ) ) ;
#73336=ORIENTED_EDGE ( 'NONE', *, *, #57573, .F. ) ;
#73337=DIRECTION ( 'NONE',  ( 0.000000000000000000, 0.000000000000000000, 1.000000000000000000 ) ) ;
#73338=ADVANCED_FACE ( 'NONE', ( #128516 ), #30854, .T. ) ;
#73339=ADVANCED_FACE ( 'NONE', ( #96426 ), #87256, .T. ) ;
#73340=CARTESIAN_POINT ( 'NONE',  ( 0.5999999999999621192, 12.50000000000000000, 0.3464101615137758494 ) ) ;
#73341=ADVANCED_FACE ( 'NONE', ( #17201 ), #66328, .T. ) ;
#73342=CARTESIAN_POINT ( 'NONE',  ( 8.749999999999957367, 2.500000000000000000, 2.065063509461097624 ) ) ;
#73343=ADVANCED_FACE ( 'NONE', ( #117334 ), #127208, .T. ) ;
#73344=DIRECTION ( 'NONE',  ( 0.000000000000000000, 0.000000000000000000, 1.000000000000000000 ) ) ;
#73345=EDGE_LOOP ( 'NONE', ( #95413, #113499, #22914, #119998 ) ) ;
#73346=EDGE_LOOP ( 'NONE', ( #121718, #118542 ) ) ;
#73347=EDGE_CURVE ( 'NONE', #106262, #9617, #7834, .T. ) ;
#73348=ORIENTED_EDGE ( 'NONE', *, *, #8063, .F. ) ;
#73349=VECTOR ( 'NONE', #108728, 1000.000000000000000 ) ;
#73350=CARTESIAN_POINT ( 'NONE',  ( -3.469446951953614189E-14, 2.500000000000000000, -0.6928203230275519209 ) ) ;
#73351=CIRCLE ( 'NONE', #75408, 0.06509327318403745899 ) ;
#73352=CONICAL_SURFACE ( 'NONE', #71211, 0.09999999999999999167, 0.003490658503988666988 ) ;
#73353=EDGE_CURVE ( 'NONE', #96049, #39206, #2094, .T. ) ;
#73354=DIRECTION ( 'NONE',  ( -0.000000000000000000, 1.000000000000000000, -0.000000000000000000 ) ) ;
#73355=CARTESIAN_POINT ( 'NONE',  ( -13.54999999999998828, 2.500000000000000000, 1.918653347947325338 ) ) ;
#73356=ADVANCED_FACE ( 'NONE', ( #110131 ), #93530, .T. ) ;
#73357=AXIS2_PLACEMENT_3D ( 'NONE', #87842, #39433, #51813 ) ;
#73358=EDGE_CURVE ( 'NONE', #19796, #87887, #12044, .T. ) ;
#73359=AXIS2_PLACEMENT_3D ( 'NONE', #42909, #12119, #50771 ) ;
#73360=VERTEX_POINT ( 'NONE', #91778 ) ;
#73361=CARTESIAN_POINT ( 'NONE',  ( 2.299999999999947864, 2.500000000000000000, 3.983716857408420964 ) ) ;
#73362=DIRECTION ( 'NONE',  ( 0.000000000000000000, 0.000000000000000000, 1.000000000000000000 ) ) ;
#73363=ADVANCED_FACE ( 'NONE', ( #42043 ), #26630, .T. ) ;
#73364=DIRECTION ( 'NONE',  ( 0.000000000000000000, 0.000000000000000000, -1.000000000000000000 ) ) ;
#73365=DIRECTION ( 'NONE',  ( 0.000000000000000000, 0.000000000000000000, -1.000000000000000000 ) ) ;
#73366=EDGE_CURVE ( 'NONE', #25430, #40175, #49632, .T. ) ;
#73367=CARTESIAN_POINT ( 'NONE',  ( -2.100000000000033840, 12.50000000000000000, 3.572213422710607489 ) ) ;
#73368=ORIENTED_EDGE ( 'NONE', *, *, #72801, .T. ) ;
#73371=LINE ( 'NONE', #44569, #14226 ) ;
#73372=DIRECTION ( 'NONE',  ( 0.000000000000000000, 1.000000000000000000, 0.000000000000000000 ) ) ;
#73373=DIRECTION ( 'NONE',  ( 0.000000000000000000, 0.000000000000000000, 1.000000000000000000 ) ) ;
#73374=DIRECTION ( 'NONE',  ( 0.000000000000000000, 0.000000000000000000, -1.000000000000000000 ) ) ;
#73375=ORIENTED_EDGE ( 'NONE', *, *, #69373, .T. ) ;
#73377=ORIENTED_EDGE ( 'NONE', *, *, #116236, .T. ) ;
#73378=DIRECTION ( 'NONE',  ( 0.000000000000000000, 1.000000000000000000, 0.000000000000000000 ) ) ;
#73379=FACE_OUTER_BOUND ( 'NONE', #31311, .T. ) ;
#73380=FACE_OUTER_BOUND ( 'NONE', #56437, .T. ) ;
#73381=DIRECTION ( 'NONE',  ( 0.000000000000000000, 0.000000000000000000, -1.000000000000000000 ) ) ;
#73382=DIRECTION ( 'NONE',  ( 0.000000000000000000, 0.000000000000000000, 1.000000000000000000 ) ) ;
#73383=EDGE_LOOP ( 'NONE', ( #98091, #50061, #82648, #82624 ) ) ;
#73384=CONICAL_SURFACE ( 'NONE', #65060, 0.1000000000000002554, 0.003490658503988666988 ) ;
#73385=DIRECTION ( 'NONE',  ( 0.000000000000000000, 0.000000000000000000, -1.000000000000000000 ) ) ;
#73386=AXIS2_PLACEMENT_3D ( 'NONE', #106481, #56080, #97945 ) ;
#73387=DIRECTION ( 'NONE',  ( 0.000000000000000000, 1.000000000000000000, 0.000000000000000000 ) ) ;
#73388=ORIENTED_EDGE ( 'NONE', *, *, #43845, .T. ) ;
#73389=DIRECTION ( 'NONE',  ( 0.000000000000000000, 0.000000000000000000, 1.000000000000000000 ) ) ;
#73390=ORIENTED_EDGE ( 'NONE', *, *, #22047, .F. ) ;
#73391=AXIS2_PLACEMENT_3D ( 'NONE', #22690, #62608, #112981 ) ;
#73392=DIRECTION ( 'NONE',  ( 0.000000000000000000, -0.000000000000000000, 1.000000000000000000 ) ) ;
#73393=CIRCLE ( 'NONE', #23222, 0.1000000000000000056 ) ;
#73394=EDGE_CURVE ( 'NONE', #8233, #51670, #118562, .T. ) ;
#73395=ORIENTED_EDGE ( 'NONE', *, *, #102634, .T. ) ;
#73396=CARTESIAN_POINT ( 'NONE',  ( -2.500000000000030642, 12.50000000000000000, -0.6928203230275541413 ) ) ;
#73397=CARTESIAN_POINT ( 'NONE',  ( 3.749999999999978684, 2.500000000000000000, -6.595190528383302109 ) ) ;
#73398=EDGE_CURVE ( 'NONE', #2346, #119558, #114448, .T. ) ;
#73399=ORIENTED_EDGE ( 'NONE', *, *, #94511, .F. ) ;
#73400=ORIENTED_EDGE ( 'NONE', *, *, #39373, .T. ) ;
#73403=AXIS2_PLACEMENT_3D ( 'NONE', #65303, #115698, #5735 ) ;
#73404=DIRECTION ( 'NONE',  ( -0.000000000000000000, 1.000000000000000000, -0.000000000000000000 ) ) ;
#73406=AXIS2_PLACEMENT_3D ( 'NONE', #56627, #78891, #9489 ) ;
#73407=CARTESIAN_POINT ( 'NONE',  ( 8.149999999999920419, 12.50000000000000000, 6.083687093685483660 ) ) ;
#73408=DIRECTION ( 'NONE',  ( 0.000000000000000000, 0.000000000000000000, 1.000000000000000000 ) ) ;
#73410=CARTESIAN_POINT ( 'NONE',  ( 6.449999999999928235, 12.50000000000000000, 2.511473670974873507 ) ) ;
#73411=CIRCLE ( 'NONE', #16948, 0.06509327318403745899 ) ;
#73412=ORIENTED_EDGE ( 'NONE', *, *, #66677, .T. ) ;
#73413=ORIENTED_EDGE ( 'NONE', *, *, #104431, .F. ) ;
#73414=CARTESIAN_POINT ( 'NONE',  ( 14.14999999999989733, 12.50000000000000000, 2.857883832488649301 ) ) ;
#73415=ORIENTED_EDGE ( 'NONE', *, *, #81203, .F. ) ;
#73416=VECTOR ( 'NONE', #536, 1000.000000000000000 ) ;
#73417=DIRECTION ( 'NONE',  ( 0.000000000000000000, 0.000000000000000000, -1.000000000000000000 ) ) ;
#73418=DIRECTION ( 'NONE',  ( 0.000000000000000000, 0.000000000000000000, 1.000000000000000000 ) ) ;
#73419=FACE_OUTER_BOUND ( 'NONE', #32666, .T. ) ;
#73420=EDGE_LOOP ( 'NONE', ( #65203, #61555, #127605, #90009 ) ) ;
#73421=ORIENTED_EDGE ( 'NONE', *, *, #114728, .F. ) ;
#73422=FACE_BOUND ( 'NONE', #268, .T. ) ;
#73423=ORIENTED_EDGE ( 'NONE', *, *, #71744, .T. ) ;
#73424=PLANE ( 'NONE',  #42956 ) ;
#73425=CARTESIAN_POINT ( 'NONE',  ( -12.89999999999999147, 12.50000000000000000, -0.6928203230275500335 ) ) ;
#73426=CARTESIAN_POINT ( 'NONE',  ( 14.34999999999989662, 2.500000000000000000, 2.511473670974873507 ) ) ;
#73427=DIRECTION ( 'NONE',  ( 0.000000000000000000, 0.000000000000000000, 1.000000000000000000 ) ) ;
#73428=DIRECTION ( 'NONE',  ( 0.000000000000000000, 0.000000000000000000, -1.000000000000000000 ) ) ;
#73429=DIRECTION ( 'NONE',  ( -0.000000000000000000, 1.000000000000000000, -0.000000000000000000 ) ) ;
#73430=CARTESIAN_POINT ( 'NONE',  ( 12.04999999999990834, 2.500000000000000000, 6.495190528383297135 ) ) ;
#73431=DIRECTION ( 'NONE',  ( -0.000000000000000000, -1.000000000000000000, -0.000000000000000000 ) ) ;
#73432=FACE_OUTER_BOUND ( 'NONE', #97635, .T. ) ;
#73433=CARTESIAN_POINT ( 'NONE',  ( 9.799999999999917222, 2.500000000000000000, 0.3464101615137735735 ) ) ;
#73434=CARTESIAN_POINT ( 'NONE',  ( 4.149999999999939959, 2.500000000000000000, -2.165063509461101710 ) ) ;
#73435=EDGE_CURVE ( 'NONE', #34432, #118817, #72151, .T. ) ;
#73436=VERTEX_POINT ( 'NONE', #121881 ) ;
#73437=ORIENTED_EDGE ( 'NONE', *, *, #100137, .F. ) ;
#73439=CARTESIAN_POINT ( 'NONE',  ( -2.900000000000030553, 12.50000000000000000, 5.088040615133786027 ) ) ;
#73440=ORIENTED_EDGE ( 'NONE', *, *, #67132, .F. ) ;
#73441=AXIS2_PLACEMENT_3D ( 'NONE', #62228, #2628, #83781 ) ;
#73442=DIRECTION ( 'NONE',  ( 0.000000000000000000, 1.000000000000000000, 0.000000000000000000 ) ) ;
#73443=CIRCLE ( 'NONE', #94372, 0.06509327318403745899 ) ;
#73444=AXIS2_PLACEMENT_3D ( 'NONE', #46763, #9415, #86672 ) ;
#73445=EDGE_LOOP ( 'NONE', ( #40199, #3550 ) ) ;
#73446=ORIENTED_EDGE ( 'NONE', *, *, #45750, .F. ) ;
#73447=EDGE_LOOP ( 'NONE', ( #3199, #104000, #13155, #17338, #76229, #117556 ) ) ;
#73448=CARTESIAN_POINT ( 'NONE',  ( -1.050000000000038680, 12.50000000000000000, 2.511473670974873507 ) ) ;
#73449=VECTOR ( 'NONE', #50356, 1000.000000000000000 ) ;
#73450=DIRECTION ( 'NONE',  ( 0.000000000000000000, -0.9999939076577903929, 0.003490651415223739937 ) ) ;
#73451=CONICAL_SURFACE ( 'NONE', #77654, 0.1000000000000002554, 0.003490658503988666988 ) ;
#73453=DIRECTION ( 'NONE',  ( -4.274815082592931898E-19, -0.9999939076577903929, -0.003490651415223739937 ) ) ;
#73454=CIRCLE ( 'NONE', #31617, 0.1000000000000000472 ) ;
#73455=EDGE_CURVE ( 'NONE', #81450, #18351, #2744, .T. ) ;
#73456=FACE_OUTER_BOUND ( 'NONE', #106175, .T. ) ;
#73457=ADVANCED_FACE ( 'NONE', ( #81324 ), #102252, .T. ) ;
#73458=EDGE_LOOP ( 'NONE', ( #78338, #108758 ) ) ;
#73459=DIRECTION ( 'NONE',  ( 0.000000000000000000, 0.000000000000000000, -1.000000000000000000 ) ) ;
#73460=EDGE_LOOP ( 'NONE', ( #76709, #102085 ) ) ;
#73461=EDGE_LOOP ( 'NONE', ( #49993, #221 ) ) ;
#73462=ORIENTED_EDGE ( 'NONE', *, *, #32460, .F. ) ;
#73463=DIRECTION ( 'NONE',  ( -0.000000000000000000, -1.000000000000000000, -0.000000000000000000 ) ) ;
#73464=EDGE_LOOP ( 'NONE', ( #102379, #49278, #80557, #113526 ) ) ;
#73465=ADVANCED_FACE ( 'NONE', ( #40774 ), #9906, .T. ) ;
#73466=ORIENTED_EDGE ( 'NONE', *, *, #78073, .F. ) ;
#73467=VERTEX_POINT ( 'NONE', #80027 ) ;
#73468=CARTESIAN_POINT ( 'NONE',  ( -4.800000000000028244, 12.50000000000000000, -3.983716857408426293 ) ) ;
#73469=DIRECTION ( 'NONE',  ( 0.000000000000000000, 0.000000000000000000, 1.000000000000000000 ) ) ;
#73470=CARTESIAN_POINT ( 'NONE',  ( -4.999999999999986677, 2.500000000000000000, 4.230127018922196669 ) ) ;
#73471=FACE_OUTER_BOUND ( 'NONE', #2944, .T. ) ;
#73472=DIRECTION ( 'NONE',  ( 0.000000000000000000, 1.000000000000000000, 0.000000000000000000 ) ) ;
#73473=CARTESIAN_POINT ( 'NONE',  ( 1.249999999999988454, 2.500000000000000000, 2.165063509461097713 ) ) ;
#73474=DIRECTION ( 'NONE',  ( 0.000000000000000000, -0.000000000000000000, 1.000000000000000000 ) ) ;
#73475=AXIS2_PLACEMENT_3D ( 'NONE', #102638, #72560, #124873 ) ;
#73476=CIRCLE ( 'NONE', #69268, 0.06509327318403745899 ) ;
#73477=ORIENTED_EDGE ( 'NONE', *, *, #126642, .T. ) ;
#73478=FACE_OUTER_BOUND ( 'NONE', #77443, .T. ) ;
#73479=ORIENTED_EDGE ( 'NONE', *, *, #103952, .F. ) ;
#73480=DIRECTION ( 'NONE',  ( 0.000000000000000000, 1.000000000000000000, 0.000000000000000000 ) ) ;
#73481=EDGE_LOOP ( 'NONE', ( #125748, #121132 ) ) ;
#73482=EDGE_LOOP ( 'NONE', ( #51889, #4339, #87305, #8164 ) ) ;
#73483=DIRECTION ( 'NONE',  ( 0.000000000000000000, 1.000000000000000000, 0.000000000000000000 ) ) ;
#73484=FACE_OUTER_BOUND ( 'NONE', #10739, .T. ) ;
#73485=CONICAL_SURFACE ( 'NONE', #79759, 0.09999999999999982514, 0.003490658503988666988 ) ;
#73486=ADVANCED_FACE ( 'NONE', ( #119297 ), #24572, .T. ) ;
#73487=CONICAL_SURFACE ( 'NONE', #33784, 0.1000000000000002554, 0.003490658503988666988 ) ;
#73488=DIRECTION ( 'NONE',  ( -0.000000000000000000, 1.000000000000000000, -0.000000000000000000 ) ) ;
#73489=EDGE_LOOP ( 'NONE', ( #30805, #92581 ) ) ;
#73490=VERTEX_POINT ( 'NONE', #91137 ) ;
#73492=FACE_OUTER_BOUND ( 'NONE', #35815, .T. ) ;
#73493=DIRECTION ( 'NONE',  ( 0.000000000000000000, 0.000000000000000000, 1.000000000000000000 ) ) ;
#73494=EDGE_CURVE ( 'NONE', #60152, #65538, #61025, .T. ) ;
#73495=CARTESIAN_POINT ( 'NONE',  ( -7.700000000000014388, 2.500000000000000000, -0.2464101615137782308 ) ) ;
#73496=DIRECTION ( 'NONE',  ( 0.000000000000000000, 0.000000000000000000, 1.000000000000000000 ) ) ;
#73497=EDGE_CURVE ( 'NONE', #49149, #123206, #50553, .T. ) ;
#73498=CONICAL_SURFACE ( 'NONE', #75637, 0.1000000000000000472, 0.003490658503988666988 ) ;
#73499=CONICAL_SURFACE ( 'NONE', #69387, 0.1000000000000000472, 0.003490658503988666988 ) ;
#73500=CARTESIAN_POINT ( 'NONE',  ( -3.150000000000033218, 2.500000000000000000, -6.841600689897078702 ) ) ;
#73501=EDGE_LOOP ( 'NONE', ( #33065, #83657 ) ) ;
#73502=VECTOR ( 'NONE', #78369, 1000.000000000000000 ) ;
#73503=EDGE_CURVE ( 'NONE', #69257, #17553, #60410, .T. ) ;
#73504=EDGE_CURVE ( 'NONE', #122281, #16616, #1455, .T. ) ;
#73505=EDGE_CURVE ( 'NONE', #11230, #48106, #124923, .T. ) ;
#73506=ORIENTED_EDGE ( 'NONE', *, *, #50755, .F. ) ;
#73507=CARTESIAN_POINT ( 'NONE',  ( -10.20000000000000284, 12.50000000000000000, -0.3464101615137782364 ) ) ;
#73508=CARTESIAN_POINT ( 'NONE',  ( -8.150000000000012790, 12.50000000000000000, -2.511473670974877948 ) ) ;
#73509=EDGE_CURVE ( 'NONE', #114154, #39901, #28788, .T. ) ;
#73510=AXIS2_PLACEMENT_3D ( 'NONE', #17194, #5462, #125880 ) ;
#73511=AXIS2_PLACEMENT_3D ( 'NONE', #1038, #61259, #19372 ) ;
#73513=DIRECTION ( 'NONE',  ( 0.000000000000000000, 0.000000000000000000, -1.000000000000000000 ) ) ;
#73514=DIRECTION ( 'NONE',  ( -0.000000000000000000, -1.000000000000000000, -0.000000000000000000 ) ) ;
#73515=CARTESIAN_POINT ( 'NONE',  ( 11.24999999999990585, 2.500000000000000000, -5.702370205355749455 ) ) ;
#73516=FACE_OUTER_BOUND ( 'NONE', #80069, .T. ) ;
#73517=ORIENTED_EDGE ( 'NONE', *, *, #28, .T. ) ;
#73519=CARTESIAN_POINT ( 'NONE',  ( 3.349999999999945466, 12.50000000000000000, -7.188010851410854052 ) ) ;
#73520=CARTESIAN_POINT ( 'NONE',  ( -13.34999999999999076, 12.50000000000000000, -1.472243186433547901 ) ) ;
#73522=ORIENTED_EDGE ( 'NONE', *, *, #17496, .F. ) ;
#73523=FACE_OUTER_BOUND ( 'NONE', #92654, .T. ) ;
#73524=ORIENTED_EDGE ( 'NONE', *, *, #55826, .F. ) ;
#73525=CARTESIAN_POINT ( 'NONE',  ( 105.5000000000000142, -1.500000000000000222, 1.322875655532295136 ) ) ;
#73526=CONICAL_SURFACE ( 'NONE', #113244, 0.09999999999999999167, 0.003490658503988666988 ) ;
#73527=AXIS2_PLACEMENT_3D ( 'NONE', #68505, #50182, #79621 ) ;
#73528=CIRCLE ( 'NONE', #88091, 0.1000000000000002554 ) ;
#73529=ORIENTED_EDGE ( 'NONE', *, *, #43979, .T. ) ;
#73530=PLANE ( 'NONE',  #29156 ) ;
#73531=CARTESIAN_POINT ( 'NONE',  ( -3.350000000000028511, 12.50000000000000000, 1.537336459617582918 ) ) ;
#73532=FACE_OUTER_BOUND ( 'NONE', #41942, .T. ) ;
#73533=ORIENTED_EDGE ( 'NONE', *, *, #6977, .T. ) ;
#73534=CONICAL_SURFACE ( 'NONE', #4471, 0.1000000000000000056, 0.003490658503988666988 ) ;
#73535=CARTESIAN_POINT ( 'NONE',  ( -7.950000000000009059, 12.50000000000000000, 6.560283801567334372 ) ) ;
#73536=AXIS2_PLACEMENT_3D ( 'NONE', #20663, #102443, #31141 ) ;
#73537=CARTESIAN_POINT ( 'NONE',  ( 3.299999999999942979, 2.500000000000000000, 4.230127018922196669 ) ) ;
#73538=AXIS2_PLACEMENT_3D ( 'NONE', #83592, #103870, #54120 ) ;
#73539=CIRCLE ( 'NONE', #17084, 0.06509327318403741736 ) ;
#73540=ORIENTED_EDGE ( 'NONE', *, *, #8893, .F. ) ;
#73541=AXIS2_PLACEMENT_3D ( 'NONE', #116230, #115577, #16082 ) ;
#73542=EDGE_CURVE ( 'NONE', #53221, #2439, #76807, .T. ) ;
#73543=ORIENTED_EDGE ( 'NONE', *, *, #82549, .T. ) ;
#73544=EDGE_LOOP ( 'NONE', ( #23477, #61637 ) ) ;
#73545=DIRECTION ( 'NONE',  ( 0.000000000000000000, 0.000000000000000000, 1.000000000000000000 ) ) ;
#73546=CARTESIAN_POINT ( 'NONE',  ( -3.749999999999994671, 12.50000000000000000, -6.495190528383302464 ) ) ;
#73547=CARTESIAN_POINT ( 'NONE',  ( -6.050000000000018474, 12.50000000000000000, 2.511473670974873507 ) ) ;
#73549=DIRECTION ( 'NONE',  ( -0.000000000000000000, -1.000000000000000000, -0.000000000000000000 ) ) ;
#73551=ORIENTED_EDGE ( 'NONE', *, *, #48720, .T. ) ;
#73552=ADVANCED_FACE ( 'NONE', ( #93712 ), #85110, .T. ) ;
#73553=CARTESIAN_POINT ( 'NONE',  ( -7.950000000000012612, 12.50000000000000000, -2.165063509461101710 ) ) ;
#73554=CARTESIAN_POINT ( 'NONE',  ( -4.999999999999990230, 2.500000000000000000, -4.330127018922201643 ) ) ;
#73555=CARTESIAN_POINT ( 'NONE',  ( 14.59999999999989484, 12.50000000000000000, -0.6928203230275541413 ) ) ;
#73556=DIRECTION ( 'NONE',  ( 0.000000000000000000, 0.000000000000000000, 1.000000000000000000 ) ) ;
#73557=DIRECTION ( 'NONE',  ( -0.000000000000000000, -1.000000000000000000, -0.000000000000000000 ) ) ;
#73558=CARTESIAN_POINT ( 'NONE',  ( -12.89999999999999147, 12.50000000000000000, -0.6277270498435125745 ) ) ;
#73559=CARTESIAN_POINT ( 'NONE',  ( -12.04999999999999538, 2.500000000000000000, 6.495190528383297135 ) ) ;
#73560=CIRCLE ( 'NONE', #59006, 0.06509327318403745899 ) ;
#73561=CIRCLE ( 'NONE', #117453, 0.06509327318403745899 ) ;
#73562=ORIENTED_EDGE ( 'NONE', *, *, #90020, .F. ) ;
#73563=VERTEX_POINT ( 'NONE', #25597 ) ;
#73564=ORIENTED_EDGE ( 'NONE', *, *, #46179, .F. ) ;
#73565=VERTEX_POINT ( 'NONE', #75347 ) ;
#73566=LINE ( 'NONE', #115404, #124837 ) ;
#73567=DIRECTION ( 'NONE',  ( 0.000000000000000000, 0.000000000000000000, 1.000000000000000000 ) ) ;
#73568=CARTESIAN_POINT ( 'NONE',  ( -5.200000000000022382, 2.500000000000000000, 0.3464101615137735735 ) ) ;
#73569=EDGE_LOOP ( 'NONE', ( #92986, #12171 ) ) ;
#73570=FACE_BOUND ( 'NONE', #26424, .T. ) ;
#73571=CONICAL_SURFACE ( 'NONE', #27596, 0.09999999999999982514, 0.003490658503988666988 ) ;
#73572=CARTESIAN_POINT ( 'NONE',  ( 12.49999999999990585, 2.500000000000000000, -5.122947341949753763 ) ) ;
#73573=DIRECTION ( 'NONE',  ( 0.000000000000000000, -0.000000000000000000, 1.000000000000000000 ) ) ;
#73574=AXIS2_PLACEMENT_3D ( 'NONE', #120158, #21300, #61242 ) ;
#73575=CONICAL_SURFACE ( 'NONE', #109069, 0.1000000000000000472, 0.003490658503988666988 ) ;
#73576=CARTESIAN_POINT ( 'NONE',  ( 3.749999999999942268, 2.500000000000000000, 1.372243186433545370 ) ) ;
#73577=CIRCLE ( 'NONE', #107017, 0.09999999999999982514 ) ;
#73578=DIRECTION ( 'NONE',  ( 0.000000000000000000, 0.000000000000000000, 1.000000000000000000 ) ) ;
#73579=DIRECTION ( 'NONE',  ( -0.000000000000000000, 1.000000000000000000, -0.000000000000000000 ) ) ;
#73580=CARTESIAN_POINT ( 'NONE',  ( 2.499999999999983569, 2.500000000000000000, -2.276824562219559311E-15 ) ) ;
#73581=DIRECTION ( 'NONE',  ( -0.000000000000000000, 1.000000000000000000, -0.000000000000000000 ) ) ;
#73582=DIRECTION ( 'NONE',  ( 0.000000000000000000, 1.000000000000000000, 0.000000000000000000 ) ) ;
#73583=DIRECTION ( 'NONE',  ( 0.000000000000000000, 0.000000000000000000, 1.000000000000000000 ) ) ;
#73585=LINE ( 'NONE', #44139, #110758 ) ;
#73586=ORIENTED_EDGE ( 'NONE', *, *, #71021, .F. ) ;
#73587=CONICAL_SURFACE ( 'NONE', #33894, 0.1000000000000002554, 0.003490658503988666988 ) ;
#73588=EDGE_CURVE ( 'NONE', #63275, #40211, #13201, .T. ) ;
#73589=ORIENTED_EDGE ( 'NONE', *, *, #119224, .F. ) ;
#73591=VERTEX_POINT ( 'NONE', #54421 ) ;
#73592=CIRCLE ( 'NONE', #27612, 0.1000000000000002554 ) ;
#73593=VERTEX_POINT ( 'NONE', #105469 ) ;
#73594=CONICAL_SURFACE ( 'NONE', #8742, 0.1000000000000002554, 0.003490658503988666988 ) ;
#73595=AXIS2_PLACEMENT_3D ( 'NONE', #96942, #24989, #34837 ) ;
#73596=EDGE_LOOP ( 'NONE', ( #66814, #49976, #349, #90445 ) ) ;
#73597=DIRECTION ( 'NONE',  ( 0.000000000000000000, 0.000000000000000000, 1.000000000000000000 ) ) ;
#73598=VERTEX_POINT ( 'NONE', #4029 ) ;
#73599=ORIENTED_EDGE ( 'NONE', *, *, #128035, .F. ) ;
#73601=EDGE_CURVE ( 'NONE', #53445, #31778, #3397, .T. ) ;
#73602=CONICAL_SURFACE ( 'NONE', #100699, 0.09999999999999982514, 0.003490658503988666988 ) ;
#73603=CARTESIAN_POINT ( 'NONE',  ( 16.56576425164984201, -1.500000000000000000, 6.084390597446049043 ) ) ;
#73605=DIRECTION ( 'NONE',  ( 0.000000000000000000, 0.000000000000000000, -1.000000000000000000 ) ) ;
#73606=EDGE_CURVE ( 'NONE', #123356, #98747, #3642, .T. ) ;
#73607=EDGE_CURVE ( 'NONE', #67054, #23927, #37107, .T. ) ;
#73608=ORIENTED_EDGE ( 'NONE', *, *, #9835, .T. ) ;
#73609=DIRECTION ( 'NONE',  ( 0.000000000000000000, -0.9999939076577903929, 0.003490651415223739937 ) ) ;
#73610=EDGE_LOOP ( 'NONE', ( #11351, #9201, #56619, #118348 ) ) ;
#73611=ORIENTED_EDGE ( 'NONE', *, *, #87672, .F. ) ;
#73612=DIRECTION ( 'NONE',  ( 0.000000000000000000, -0.000000000000000000, 1.000000000000000000 ) ) ;
#73613=ORIENTED_EDGE ( 'NONE', *, *, #36547, .T. ) ;
#73614=EDGE_CURVE ( 'NONE', #106514, #79569, #64879, .T. ) ;
#73615=CARTESIAN_POINT ( 'NONE',  ( 9.599999999999917932, 2.500000000000000000, 0.5928203230275495006 ) ) ;
#73616=EDGE_CURVE ( 'NONE', #54834, #80090, #14180, .T. ) ;
#73617=VERTEX_POINT ( 'NONE', #23043 ) ;
#73618=FACE_OUTER_BOUND ( 'NONE', #66928, .T. ) ;
#73619=CARTESIAN_POINT ( 'NONE',  ( -8.749999999999975131, 2.500000000000000000, -2.265063509461101798 ) ) ;
#73620=CARTESIAN_POINT ( 'NONE',  ( 5.849999999999932143, 2.500000000000000000, 1.372243186433545370 ) ) ;
#73621=AXIS2_PLACEMENT_3D ( 'NONE', #50869, #69200, #71142 ) ;
#73622=DIRECTION ( 'NONE',  ( -0.000000000000000000, -1.000000000000000000, -0.000000000000000000 ) ) ;
#73623=AXIS2_PLACEMENT_3D ( 'NONE', #90327, #60887, #674 ) ;
#73624=CARTESIAN_POINT ( 'NONE',  ( -1.250000000000037970, 2.500000000000000000, 2.857883832488649301 ) ) ;
#73625=ORIENTED_EDGE ( 'NONE', *, *, #121835, .T. ) ;
#73626=DIRECTION ( 'NONE',  ( 0.000000000000000000, 1.000000000000000000, 0.000000000000000000 ) ) ;
#73627=AXIS2_PLACEMENT_3D ( 'NONE', #58738, #18797, #31696 ) ;
#73628=CIRCLE ( 'NONE', #8782, 0.1000000000000000472 ) ;
#73629=ORIENTED_EDGE ( 'NONE', *, *, #127884, .F. ) ;
#73630=CARTESIAN_POINT ( 'NONE',  ( 17.50000000000000000, 2.499999999999999556, -1.666666666666663410 ) ) ;
#73631=CIRCLE ( 'NONE', #50659, 0.1000000000000002554 ) ;
#73632=EDGE_LOOP ( 'NONE', ( #123554, #122454 ) ) ;
#73633=CARTESIAN_POINT ( 'NONE',  ( 2.049999999999950084, 2.500000000000000000, -6.495190528383302464 ) ) ;
#73634=DIRECTION ( 'NONE',  ( 0.000000000000000000, -0.9999939076577903929, 0.003490651415223739937 ) ) ;
#73635=CIRCLE ( 'NONE', #54847, 0.06509327318403745899 ) ;
#73636=CARTESIAN_POINT ( 'NONE',  ( 6.049999999999934097, 2.500000000000000000, 6.048780366869521252 ) ) ;
#73637=DIRECTION ( 'NONE',  ( -0.000000000000000000, 1.000000000000000000, -0.000000000000000000 ) ) ;
#73638=EDGE_LOOP ( 'NONE', ( #51650, #20651, #35763, #49407 ) ) ;
#73639=CIRCLE ( 'NONE', #119612, 0.1000000000000002554 ) ;
#73640=FACE_OUTER_BOUND ( 'NONE', #124142, .T. ) ;
#73641=CARTESIAN_POINT ( 'NONE',  ( -4.200000000000025935, 12.50000000000000000, 4.330127018922196314 ) ) ;
#73642=ORIENTED_EDGE ( 'NONE', *, *, #112374, .F. ) ;
#73644=ORIENTED_EDGE ( 'NONE', *, *, #70522, .T. ) ;
#73645=DIRECTION ( 'NONE',  ( 0.000000000000000000, 0.000000000000000000, 1.000000000000000000 ) ) ;
#73646=DIRECTION ( 'NONE',  ( 0.000000000000000000, -0.000000000000000000, 1.000000000000000000 ) ) ;
#73648=DIRECTION ( 'NONE',  ( 0.000000000000000000, 0.000000000000000000, -1.000000000000000000 ) ) ;
#73649=ADVANCED_FACE ( 'NONE', ( #24331 ), #24969, .T. ) ;
#73650=CARTESIAN_POINT ( 'NONE',  ( 17.27571223834410219, 2.230085210383166316, -5.047251339834024186 ) ) ;
#73651=DIRECTION ( 'NONE',  ( -4.274815082592931898E-19, -0.9999939076577903929, -0.003490651415223739937 ) ) ;
#73652=EDGE_CURVE ( 'NONE', #41483, #54886, #5318, .T. ) ;
#73653=EDGE_CURVE ( 'NONE', #33436, #73847, #37197, .T. ) ;
#73654=ADVANCED_FACE ( 'NONE', ( #5954 ), #16228, .T. ) ;
#73655=AXIS2_PLACEMENT_3D ( 'NONE', #76265, #116167, #26516 ) ;
#73656=ORIENTED_EDGE ( 'NONE', *, *, #70036, .T. ) ;
#73657=CARTESIAN_POINT ( 'NONE',  ( 11.84999999999990727, 2.500000000000000000, -2.511473670974877948 ) ) ;
#73658=AXIS2_PLACEMENT_3D ( 'NONE', #1043, #92006, #381 ) ;
#73660=EDGE_CURVE ( 'NONE', #39039, #37067, #70633, .T. ) ;
#73661=DIRECTION ( 'NONE',  ( 0.000000000000000000, -0.9999939076577903929, 0.003490651415223739937 ) ) ;
#73662=LINE ( 'NONE', #94588, #60097 ) ;
#73663=DIRECTION ( 'NONE',  ( -0.000000000000000000, -1.000000000000000000, -0.000000000000000000 ) ) ;
#73664=CARTESIAN_POINT ( 'NONE',  ( -6.450000000000014388, 12.50000000000000000, 1.818653347947321475 ) ) ;
#73665=CIRCLE ( 'NONE', #27695, 0.06509327318403745899 ) ;
#73666=ORIENTED_EDGE ( 'NONE', *, *, #15762, .T. ) ;
#73667=ADVANCED_FACE ( 'NONE', ( #63618 ), #74844, .T. ) ;
#73668=CIRCLE ( 'NONE', #50691, 0.06509327318403745899 ) ;
#73669=EDGE_CURVE ( 'NONE', #81872, #44930, #24669, .T. ) ;
#73670=AXIS2_PLACEMENT_3D ( 'NONE', #73507, #2843, #34907 ) ;
#73672=CARTESIAN_POINT ( 'NONE',  ( 8.349999999999919709, 2.500000000000000000, 7.288010851410849256 ) ) ;
#73673=ORIENTED_EDGE ( 'NONE', *, *, #97039, .F. ) ;
#73674=VECTOR ( 'NONE', #107348, 1000.000000000000000 ) ;
#73675=VERTEX_POINT ( 'NONE', #18363 ) ;
#73676=LINE ( 'NONE', #63224, #126190 ) ;
#73677=ORIENTED_EDGE ( 'NONE', *, *, #128557, .F. ) ;
#73678=AXIS2_PLACEMENT_3D ( 'NONE', #124352, #94883, #5197 ) ;
#73679=AXIS2_PLACEMENT_3D ( 'NONE', #98909, #9247, #49196 ) ;
#73680=ORIENTED_EDGE ( 'NONE', *, *, #40155, .F. ) ;
#73681=AXIS2_PLACEMENT_3D ( 'NONE', #19018, #119813, #98878 ) ;
#73682=DIRECTION ( 'NONE',  ( 0.000000000000000000, 0.000000000000000000, -1.000000000000000000 ) ) ;
#73683=CIRCLE ( 'NONE', #59141, 0.1000000000000002554 ) ;
#73684=EDGE_LOOP ( 'NONE', ( #125133, #124885, #83029, #104654 ) ) ;
#73685=CARTESIAN_POINT ( 'NONE',  ( 16.68526679984143613, 0.4774970013437123129, -5.954360761636884547 ) ) ;
#73686=DIRECTION ( 'NONE',  ( -0.000000000000000000, -1.000000000000000000, -0.000000000000000000 ) ) ;
#73687=DIRECTION ( 'NONE',  ( -4.274815082592931898E-19, -0.9999939076577903929, -0.003490651415223739937 ) ) ;
#73688=ORIENTED_EDGE ( 'NONE', *, *, #11201, .T. ) ;
#73689=CIRCLE ( 'NONE', #17240, 0.06509327318403745899 ) ;
#73690=DIRECTION ( 'NONE',  ( 0.000000000000000000, -0.9999939076577903929, 0.003490651415223739937 ) ) ;
#73691=DIRECTION ( 'NONE',  ( 0.000000000000000000, 0.000000000000000000, 1.000000000000000000 ) ) ;
#73692=VERTEX_POINT ( 'NONE', #36742 ) ;
#73693=DIRECTION ( 'NONE',  ( 0.000000000000000000, 0.000000000000000000, -1.000000000000000000 ) ) ;
#73694=CARTESIAN_POINT ( 'NONE',  ( -9.600000000000006750, 2.500000000000000000, -0.6928203230275542523 ) ) ;
#73695=VERTEX_POINT ( 'NONE', #125726 ) ;
#73696=ORIENTED_EDGE ( 'NONE', *, *, #23388, .T. ) ;
#73698=VERTEX_POINT ( 'NONE', #7241 ) ;
#73699=FACE_OUTER_BOUND ( 'NONE', #79819, .T. ) ;
#73700=FACE_OUTER_BOUND ( 'NONE', #101831, .T. ) ;
#73701=DIRECTION ( 'NONE',  ( 0.000000000000000000, -0.000000000000000000, 1.000000000000000000 ) ) ;
#73702=AXIS2_PLACEMENT_3D ( 'NONE', #78674, #49221, #26991 ) ;
#73703=FACE_BOUND ( 'NONE', #19617, .T. ) ;
#73704=ORIENTED_EDGE ( 'NONE', *, *, #53564, .T. ) ;
#73706=DIRECTION ( 'NONE',  ( 0.000000000000000000, 1.000000000000000000, 0.000000000000000000 ) ) ;
#73707=DIRECTION ( 'NONE',  ( -4.274815082592931898E-19, -0.9999939076577903929, -0.003490651415223739937 ) ) ;
#73708=EDGE_CURVE ( 'NONE', #41461, #120619, #96922, .T. ) ;
#73709=AXIS2_PLACEMENT_3D ( 'NONE', #29783, #118803, #48790 ) ;
#73710=VECTOR ( 'NONE', #75218, 1000.000000000000000 ) ;
#73711=CARTESIAN_POINT ( 'NONE',  ( 5.649999999999934630, 2.500000000000000000, 6.941600689897073018 ) ) ;
#73712=AXIS2_PLACEMENT_3D ( 'NONE', #110353, #76552, #80260 ) ;
#73713=CARTESIAN_POINT ( 'NONE',  ( -14.39999999999998614, 12.50000000000000000, 0.3464101615137758494 ) ) ;
#73714=CARTESIAN_POINT ( 'NONE',  ( -1.850000000000033396, 2.500000000000000000, -6.248780366869526759 ) ) ;
#73715=AXIS2_PLACEMENT_3D ( 'NONE', #122946, #82387, #91547 ) ;
#73716=DIRECTION ( 'NONE',  ( 0.000000000000000000, -0.9999939076577903929, 0.003490651415223739937 ) ) ;
#73717=CIRCLE ( 'NONE', #102974, 0.06509327318403745899 ) ;
#73718=ORIENTED_EDGE ( 'NONE', *, *, #26059, .F. ) ;
#73719=ORIENTED_EDGE ( 'NONE', *, *, #23081, .T. ) ;
#73720=ORIENTED_EDGE ( 'NONE', *, *, #100405, .F. ) ;
#73721=ORIENTED_EDGE ( 'NONE', *, *, #24579, .F. ) ;
#73722=AXIS2_PLACEMENT_3D ( 'NONE', #61720, #49974, #30330 ) ;
#73723=ORIENTED_EDGE ( 'NONE', *, *, #95489, .F. ) ;
#73724=DIRECTION ( 'NONE',  ( 0.000000000000000000, 0.000000000000000000, 1.000000000000000000 ) ) ;
#73725=AXIS2_PLACEMENT_3D ( 'NONE', #92805, #10989, #43079 ) ;
#73726=CIRCLE ( 'NONE', #40609, 0.06509327318403745899 ) ;
#73728=ORIENTED_EDGE ( 'NONE', *, *, #113745, .F. ) ;
#73729=FACE_BOUND ( 'NONE', #127246, .T. ) ;
#73730=CARTESIAN_POINT ( 'NONE',  ( 3.149999999999946176, 2.500000000000000000, -2.611473670974877592 ) ) ;
#73732=CARTESIAN_POINT ( 'NONE',  ( 0.3999999999999563904, 2.500000000000000000, 3.637306695894644726 ) ) ;
#73733=DIRECTION ( 'NONE',  ( 0.000000000000000000, 1.000000000000000000, 0.000000000000000000 ) ) ;
#73734=CARTESIAN_POINT ( 'NONE',  ( -11.84999999999999787, 2.500000000000000000, -1.918653347947322008 ) ) ;
#73735=ORIENTED_EDGE ( 'NONE', *, *, #29737, .F. ) ;
#73736=DIRECTION ( 'NONE',  ( 0.000000000000000000, 0.000000000000000000, 1.000000000000000000 ) ) ;
#73737=VECTOR ( 'NONE', #25888, 1000.000000000000000 ) ;
#73738=EDGE_LOOP ( 'NONE', ( #88547, #47245 ) ) ;
#73739=ORIENTED_EDGE ( 'NONE', *, *, #35024, .F. ) ;
#73740=VERTEX_POINT ( 'NONE', #96269 ) ;
#73741=DIRECTION ( 'NONE',  ( 0.000000000000000000, -0.9999939076577903929, 0.003490651415223739937 ) ) ;
#73742=CARTESIAN_POINT ( 'NONE',  ( -10.20000000000000284, 2.500000000000000000, -0.3464101615137782364 ) ) ;
#73743=DIRECTION ( 'NONE',  ( -0.000000000000000000, 1.000000000000000000, -0.000000000000000000 ) ) ;
#73744=VERTEX_POINT ( 'NONE', #58315 ) ;
#73745=CARTESIAN_POINT ( 'NONE',  ( -8.350000000000012079, 2.500000000000000000, 1.472243186433545459 ) ) ;
#73746=VECTOR ( 'NONE', #82048, 1000.000000000000000 ) ;
#73747=EDGE_CURVE ( 'NONE', #15359, #33584, #18404, .T. ) ;
#73748=AXIS2_PLACEMENT_3D ( 'NONE', #81947, #63616, #11919 ) ;
#73749=LINE ( 'NONE', #124806, #7175 ) ;
#73750=FACE_OUTER_BOUND ( 'NONE', #18466, .T. ) ;
#73752=VERTEX_POINT ( 'NONE', #47197 ) ;
#73753=EDGE_CURVE ( 'NONE', #94819, #119696, #117840, .T. ) ;
#73754=DIRECTION ( 'NONE',  ( 0.000000000000000000, 1.000000000000000000, 0.000000000000000000 ) ) ;
#73755=CONICAL_SURFACE ( 'NONE', #92542, 0.1000000000000000472, 0.003490658503988666988 ) ;
#73756=ADVANCED_FACE ( 'NONE', ( #6578 ), #7928, .T. ) ;
#73757=EDGE_LOOP ( 'NONE', ( #80863, #99612 ) ) ;
#73759=CIRCLE ( 'NONE', #17305, 0.06509327318403745899 ) ;
#73760=VECTOR ( 'NONE', #66189, 1000.000000000000000 ) ;
#73761=ORIENTED_EDGE ( 'NONE', *, *, #1792, .F. ) ;
#73762=CONICAL_SURFACE ( 'NONE', #42493, 0.1000000000000002554, 0.003490658503988666988 ) ;
#73763=ORIENTED_EDGE ( 'NONE', *, *, #28279, .F. ) ;
#73764=DIRECTION ( 'NONE',  ( 0.000000000000000000, 0.000000000000000000, 1.000000000000000000 ) ) ;
#73765=DIRECTION ( 'NONE',  ( -0.000000000000000000, -1.000000000000000000, -0.000000000000000000 ) ) ;
#73766=EDGE_CURVE ( 'NONE', #105454, #37559, #38684, .T. ) ;
#73767=EDGE_CURVE ( 'NONE', #8482, #71296, #97570, .T. ) ;
#73768=CARTESIAN_POINT ( 'NONE',  ( 0.3999999999999568345, 12.50000000000000000, -5.022947341949754119 ) ) ;
#73769=EDGE_CURVE ( 'NONE', #49114, #12584, #101940, .T. ) ;
#73770=CARTESIAN_POINT ( 'NONE',  ( 7.049999999999928768, 2.500000000000000000, -2.165063509461101710 ) ) ;
#73771=EDGE_CURVE ( 'NONE', #2492, #110412, #68106, .T. ) ;
#73772=DIRECTION ( 'NONE',  ( -0.000000000000000000, -1.000000000000000000, -0.000000000000000000 ) ) ;
#73773=AXIS2_PLACEMENT_3D ( 'NONE', #26074, #117000, #5125 ) ;
#73774=VERTEX_POINT ( 'NONE', #47847 ) ;
#73775=EDGE_LOOP ( 'NONE', ( #47289, #129278 ) ) ;
#73778=CIRCLE ( 'NONE', #71738, 0.06509327318403745899 ) ;
#73779=CONICAL_SURFACE ( 'NONE', #86287, 0.1000000000000002554, 0.003490658503988666988 ) ;
#73780=DIRECTION ( 'NONE',  ( 0.000000000000000000, 0.000000000000000000, 1.000000000000000000 ) ) ;
#73781=ORIENTED_EDGE ( 'NONE', *, *, #11695, .F. ) ;
#73782=EDGE_LOOP ( 'NONE', ( #127578, #66392 ) ) ;
#73783=EDGE_CURVE ( 'NONE', #44204, #125682, #102035, .T. ) ;
#73784=DIRECTION ( 'NONE',  ( -0.000000000000000000, 1.000000000000000000, -0.000000000000000000 ) ) ;
#73785=VECTOR ( 'NONE', #120901, 1000.000000000000000 ) ;
#73786=ORIENTED_EDGE ( 'NONE', *, *, #19400, .T. ) ;
#73787=CARTESIAN_POINT ( 'NONE',  ( -3.100000000000028955, 2.500000000000000000, 3.983716857408420964 ) ) ;
#73788=LINE ( 'NONE', #103907, #40673 ) ;
#73789=VERTEX_POINT ( 'NONE', #28847 ) ;
#73790=AXIS2_PLACEMENT_3D ( 'NONE', #77135, #36587, #39172 ) ;
#73791=CARTESIAN_POINT ( 'NONE',  ( -6.650000000000018119, 2.500000000000000000, -6.495190528383302464 ) ) ;
#73792=DIRECTION ( 'NONE',  ( 0.000000000000000000, -0.000000000000000000, 1.000000000000000000 ) ) ;
#73793=PLANE ( 'NONE',  #126221 ) ;
#73794=CARTESIAN_POINT ( 'NONE',  ( 14.34999999999989662, 12.50000000000000000, 1.883746621131358934 ) ) ;
#73795=ORIENTED_EDGE ( 'NONE', *, *, #55250, .T. ) ;
#73796=CARTESIAN_POINT ( 'NONE',  ( -5.400000000000019895, 2.500000000000000000, -0.7928203230275542301 ) ) ;
#73797=CARTESIAN_POINT ( 'NONE',  ( 35.04009662963670735, -1.562391656607243329, 4.793251516052316141 ) ) ;
#73798=ORIENTED_EDGE ( 'NONE', *, *, #78583, .F. ) ;
#73799=ORIENTED_EDGE ( 'NONE', *, *, #123589, .T. ) ;
#73800=CONICAL_SURFACE ( 'NONE', #31969, 0.1000000000000002554, 0.003490658503988666988 ) ;
#73801=AXIS2_PLACEMENT_3D ( 'NONE', #115173, #25518, #83804 ) ;
#73802=ADVANCED_FACE ( 'NONE', ( #48478 ), #41405, .T. ) ;
#73804=DIRECTION ( 'NONE',  ( -0.000000000000000000, 1.000000000000000000, -0.000000000000000000 ) ) ;
#73805=DIRECTION ( 'NONE',  ( -0.000000000000000000, 1.000000000000000000, -0.000000000000000000 ) ) ;
#73806=DIRECTION ( 'NONE',  ( 0.000000000000000000, 0.000000000000000000, -1.000000000000000000 ) ) ;
#73807=CARTESIAN_POINT ( 'NONE',  ( 9.599999999999917932, 2.500000000000000000, -0.5928203230275541635 ) ) ;
#73808=AXIS2_PLACEMENT_3D ( 'NONE', #6856, #87367, #108304 ) ;
#73809=DIRECTION ( 'NONE',  ( -0.000000000000000000, 1.000000000000000000, -0.000000000000000000 ) ) ;
#73810=DIRECTION ( 'NONE',  ( -0.000000000000000000, 1.000000000000000000, -0.000000000000000000 ) ) ;
#73811=AXIS2_PLACEMENT_3D ( 'NONE', #71982, #11756, #119777 ) ;
#73812=DIRECTION ( 'NONE',  ( 0.000000000000000000, 1.000000000000000000, 0.000000000000000000 ) ) ;
#73813=FACE_OUTER_BOUND ( 'NONE', #91140, .T. ) ;
#73814=DIRECTION ( 'NONE',  ( 0.000000000000000000, 0.000000000000000000, 1.000000000000000000 ) ) ;
#73815=CIRCLE ( 'NONE', #115560, 0.06509327318403745899 ) ;
#73816=CONICAL_SURFACE ( 'NONE', #46628, 0.1000000000000000472, 0.003490658503988666988 ) ;
#73817=EDGE_CURVE ( 'NONE', #96053, #60531, #30939, .T. ) ;
#73818=ADVANCED_FACE ( 'NONE', ( #98857 ), #12129, .T. ) ;
#73819=EDGE_CURVE ( 'NONE', #43127, #27663, #78604, .T. ) ;
#73820=DIRECTION ( 'NONE',  ( 0.000000000000000000, 0.000000000000000000, -1.000000000000000000 ) ) ;
#73821=ORIENTED_EDGE ( 'NONE', *, *, #116654, .F. ) ;
#73822=VECTOR ( 'NONE', #20401, 1000.000000000000000 ) ;
#73823=VERTEX_POINT ( 'NONE', #117181 ) ;
#73824=CONICAL_SURFACE ( 'NONE', #61315, 0.1000000000000000472, 0.003490658503988666988 ) ;
#73825=EDGE_CURVE ( 'NONE', #37559, #116756, #114534, .T. ) ;
#73826=CONICAL_SURFACE ( 'NONE', #69622, 0.1000000000000002554, 0.003490658503988666988 ) ;
#73827=EDGE_LOOP ( 'NONE', ( #55650, #47510, #90060, #2559 ) ) ;
#73828=VECTOR ( 'NONE', #102586, 1000.000000000000000 ) ;
#73829=ADVANCED_FACE ( 'NONE', ( #75998 ), #115925, .T. ) ;
#73830=ORIENTED_EDGE ( 'NONE', *, *, #5937, .F. ) ;
#73831=EDGE_CURVE ( 'NONE', #79117, #18510, #120810, .T. ) ;
#73832=CARTESIAN_POINT ( 'NONE',  ( 13.09999999999989839, 2.500000000000000000, 0.3464101615137735735 ) ) ;
#73833=PLANE ( 'NONE',  #72964 ) ;
#73834=CONICAL_SURFACE ( 'NONE', #117727, 0.09999999999999982514, 0.003490658503988666988 ) ;
#73835=EDGE_CURVE ( 'NONE', #5090, #38024, #66423, .T. ) ;
#73836=ORIENTED_EDGE ( 'NONE', *, *, #14908, .F. ) ;
#73837=ADVANCED_FACE ( 'NONE', ( #11113 ), #89418, .T. ) ;
#73838=CARTESIAN_POINT ( 'NONE',  ( 1.449999999999951328, 12.50000000000000000, -1.818653347947326138 ) ) ;
#73839=EDGE_CURVE ( 'NONE', #50581, #128585, #20952, .T. ) ;
#73840=FACE_OUTER_BOUND ( 'NONE', #106382, .T. ) ;
#73841=DIRECTION ( 'NONE',  ( -0.000000000000000000, -1.000000000000000000, -0.000000000000000000 ) ) ;
#73842=VERTEX_POINT ( 'NONE', #59616 ) ;
#73843=FACE_OUTER_BOUND ( 'NONE', #118726, .T. ) ;
#73844=EDGE_CURVE ( 'NONE', #77757, #128842, #76897, .T. ) ;
#73845=CARTESIAN_POINT ( 'NONE',  ( 13.34999999999989662, 12.50000000000000000, -2.922977105672691422 ) ) ;
#73846=ORIENTED_EDGE ( 'NONE', *, *, #86803, .F. ) ;
#73847=VERTEX_POINT ( 'NONE', #101449 ) ;
#73848=ORIENTED_EDGE ( 'NONE', *, *, #14574, .T. ) ;
#73849=ORIENTED_EDGE ( 'NONE', *, *, #66943, .F. ) ;
#73850=CARTESIAN_POINT ( 'NONE',  ( 4.149999999999941735, 2.500000000000000000, -1.572243186433550211 ) ) ;
#73851=DIRECTION ( 'NONE',  ( -0.000000000000000000, -1.000000000000000000, -0.000000000000000000 ) ) ;
#73852=CARTESIAN_POINT ( 'NONE',  ( 12.69999999999989981, 12.50000000000000000, -0.3464101615137783474 ) ) ;
#73853=CARTESIAN_POINT ( 'NONE',  ( 11.04999999999990834, 12.50000000000000000, 1.818653347947321475 ) ) ;
#73854=CIRCLE ( 'NONE', #59211, 0.06509327318403743123 ) ;
#73855=VERTEX_POINT ( 'NONE', #9841 ) ;
#73856=CARTESIAN_POINT ( 'NONE',  ( -7.500000000000013323, 2.500000000000000000, 4.922947341949748257 ) ) ;
#73857=ORIENTED_EDGE ( 'NONE', *, *, #73186, .F. ) ;
#73858=CARTESIAN_POINT ( 'NONE',  ( -3.950000000000024603, 2.500000000000000000, -2.511473670974877948 ) ) ;
#73859=CARTESIAN_POINT ( 'NONE',  ( 10.04522989421447043, -2.499999999999999556, -8.164691043409833426 ) ) ;
#73860=DIRECTION ( 'NONE',  ( -4.274815082592931898E-19, -0.9999939076577903929, -0.003490651415223739937 ) ) ;
#73861=LINE ( 'NONE', #43783, #119544 ) ;
#73862=EDGE_CURVE ( 'NONE', #15192, #10596, #45609, .T. ) ;
#73863=AXIS2_PLACEMENT_3D ( 'NONE', #24145, #83712, #33339 ) ;
#73864=AXIS2_PLACEMENT_3D ( 'NONE', #86178, #44340, #114367 ) ;
#73865=CIRCLE ( 'NONE', #67588, 0.06509327318403745899 ) ;
#73866=ORIENTED_EDGE ( 'NONE', *, *, #12141, .T. ) ;
#73867=AXIS2_PLACEMENT_3D ( 'NONE', #99293, #64823, #128104 ) ;
#73868=VERTEX_POINT ( 'NONE', #1940 ) ;
#73869=VERTEX_POINT ( 'NONE', #81165 ) ;
#73870=DIRECTION ( 'NONE',  ( 0.000000000000000000, -0.9999939076577903929, 0.003490651415223739937 ) ) ;
#73871=DIRECTION ( 'NONE',  ( 0.000000000000000000, -0.000000000000000000, 1.000000000000000000 ) ) ;
#73872=DIRECTION ( 'NONE',  ( 0.000000000000000000, 0.000000000000000000, 1.000000000000000000 ) ) ;
#73873=FACE_BOUND ( 'NONE', #54097, .T. ) ;
#73874=AXIS2_PLACEMENT_3D ( 'NONE', #88382, #27530, #106742 ) ;
#73875=CARTESIAN_POINT ( 'NONE',  ( -0.8500000000000386136, 2.500000000000000000, 7.188010851410848723 ) ) ;
#73876=DIRECTION ( 'NONE',  ( 0.000000000000000000, -0.000000000000000000, 1.000000000000000000 ) ) ;
#73877=LINE ( 'NONE', #113811, #70852 ) ;
#73878=ADVANCED_FACE ( 'NONE', ( #11769 ), #72698, .T. ) ;
#73879=VECTOR ( 'NONE', #10146, 1000.000000000000000 ) ;
#73880=AXIS2_PLACEMENT_3D ( 'NONE', #14060, #114222, #85403 ) ;
#73881=AXIS2_PLACEMENT_3D ( 'NONE', #21454, #101317, #51576 ) ;
#73882=DIRECTION ( 'NONE',  ( -0.000000000000000000, -1.000000000000000000, -0.000000000000000000 ) ) ;
#73883=DIRECTION ( 'NONE',  ( 0.000000000000000000, 1.000000000000000000, 0.000000000000000000 ) ) ;
#73884=AXIS2_PLACEMENT_3D ( 'NONE', #87412, #99839, #7562 ) ;
#73885=DIRECTION ( 'NONE',  ( -0.000000000000000000, 1.000000000000000000, -0.000000000000000000 ) ) ;
#73886=VERTEX_POINT ( 'NONE', #120443 ) ;
#73887=DIRECTION ( 'NONE',  ( 0.000000000000000000, -0.9999939076577903929, 0.003490651415223739937 ) ) ;
#73888=ORIENTED_EDGE ( 'NONE', *, *, #80038, .T. ) ;
#73889=ORIENTED_EDGE ( 'NONE', *, *, #64167, .T. ) ;
#73891=ORIENTED_EDGE ( 'NONE', *, *, #54505, .T. ) ;
#73892=EDGE_CURVE ( 'NONE', #74692, #115125, #93624, .T. ) ;
#73893=DIRECTION ( 'NONE',  ( 0.000000000000000000, 1.000000000000000000, 0.000000000000000000 ) ) ;
#73894=FACE_BOUND ( 'NONE', #98339, .T. ) ;
#73895=DIRECTION ( 'NONE',  ( 0.000000000000000000, 0.000000000000000000, 1.000000000000000000 ) ) ;
#73896=AXIS2_PLACEMENT_3D ( 'NONE', #67992, #69274, #107924 ) ;
#73897=VERTEX_POINT ( 'NONE', #89690 ) ;
#73898=DIRECTION ( 'NONE',  ( 0.000000000000000000, 0.000000000000000000, 1.000000000000000000 ) ) ;
#73899=AXIS2_PLACEMENT_3D ( 'NONE', #80447, #41186, #121005 ) ;
#73900=DIRECTION ( 'NONE',  ( 0.000000000000000000, 1.000000000000000000, 0.000000000000000000 ) ) ;
#73901=ORIENTED_EDGE ( 'NONE', *, *, #118102, .F. ) ;
#73902=DIRECTION ( 'NONE',  ( -0.000000000000000000, 1.000000000000000000, -0.000000000000000000 ) ) ;
#73903=DIRECTION ( 'NONE',  ( -0.000000000000000000, -1.000000000000000000, -0.000000000000000000 ) ) ;
#73904=CIRCLE ( 'NONE', #38323, 0.06509327318403745899 ) ;
#73905=AXIS2_PLACEMENT_3D ( 'NONE', #100845, #44352, #104565 ) ;
#73906=CIRCLE ( 'NONE', #67639, 0.06509327318403745899 ) ;
#73907=AXIS2_PLACEMENT_3D ( 'NONE', #35163, #105819, #75071 ) ;
#73908=AXIS2_PLACEMENT_3D ( 'NONE', #51309, #81405, #121312 ) ;
#73909=EDGE_LOOP ( 'NONE', ( #88504, #16051, #116994, #79423 ) ) ;
#73910=DIRECTION ( 'NONE',  ( 0.000000000000000000, 0.000000000000000000, -1.000000000000000000 ) ) ;
#73911=DIRECTION ( 'NONE',  ( 0.000000000000000000, -0.000000000000000000, 1.000000000000000000 ) ) ;
#73912=AXIS2_PLACEMENT_3D ( 'NONE', #45840, #85747, #36677 ) ;
#73913=AXIS2_PLACEMENT_3D ( 'NONE', #79432, #110800, #58509 ) ;
#73914=VERTEX_POINT ( 'NONE', #109327 ) ;
#73915=CIRCLE ( 'NONE', #2916, 0.1000000000000002554 ) ;
#73916=ADVANCED_FACE ( 'NONE', ( #79239 ), #21597, .T. ) ;
#73917=DIRECTION ( 'NONE',  ( 0.000000000000000000, 0.000000000000000000, 1.000000000000000000 ) ) ;
#73918=CARTESIAN_POINT ( 'NONE',  ( 5.649999999999934630, 2.500000000000000000, 6.841600689897072485 ) ) ;
#73919=DIRECTION ( 'NONE',  ( -0.000000000000000000, -1.000000000000000000, -0.000000000000000000 ) ) ;
#73920=AXIS2_PLACEMENT_3D ( 'NONE', #123081, #94906, #103443 ) ;
#73921=ORIENTED_EDGE ( 'NONE', *, *, #102912, .F. ) ;
#73922=ORIENTED_EDGE ( 'NONE', *, *, #73358, .T. ) ;
#73923=CARTESIAN_POINT ( 'NONE',  ( 4.149999999999939959, 12.50000000000000000, -6.560283801567339701 ) ) ;
#73924=EDGE_CURVE ( 'NONE', #11458, #87465, #32999, .T. ) ;
#73925=ORIENTED_EDGE ( 'NONE', *, *, #77661, .T. ) ;
#73926=DIRECTION ( 'NONE',  ( 0.000000000000000000, 0.000000000000000000, 1.000000000000000000 ) ) ;
#73927=CARTESIAN_POINT ( 'NONE',  ( 8.349999999999923261, 2.500000000000000000, 1.472243186433545459 ) ) ;
#73928=ORIENTED_EDGE ( 'NONE', *, *, #21191, .T. ) ;
#73929=DIRECTION ( 'NONE',  ( -0.000000000000000000, -1.000000000000000000, -0.000000000000000000 ) ) ;
#73930=DIRECTION ( 'NONE',  ( 0.000000000000000000, 1.000000000000000000, 0.000000000000000000 ) ) ;
#73931=DIRECTION ( 'NONE',  ( 0.000000000000000000, 1.000000000000000000, 0.000000000000000000 ) ) ;
#73932=ADVANCED_FACE ( 'NONE', ( #51075 ), #31047, .T. ) ;
#73933=EDGE_CURVE ( 'NONE', #110796, #60290, #81788, .T. ) ;
#73934=DIRECTION ( 'NONE',  ( 0.000000000000000000, 0.000000000000000000, 1.000000000000000000 ) ) ;
#73935=EDGE_CURVE ( 'NONE', #107586, #91772, #22263, .T. ) ;
#73936=EDGE_CURVE ( 'NONE', #91958, #56615, #119793, .T. ) ;
#73937=ADVANCED_FACE ( 'NONE', ( #109982 ), #89051, .T. ) ;
#73938=DIRECTION ( 'NONE',  ( 0.000000000000000000, 1.000000000000000000, 0.000000000000000000 ) ) ;
#73939=CIRCLE ( 'NONE', #113753, 0.06509327318403745899 ) ;
#73940=EDGE_LOOP ( 'NONE', ( #61563, #70087, #8260, #96022 ) ) ;
#73941=VERTEX_POINT ( 'NONE', #119149 ) ;
#73942=DIRECTION ( 'NONE',  ( 0.000000000000000000, 1.000000000000000000, 0.000000000000000000 ) ) ;
#73943=DIRECTION ( 'NONE',  ( -4.274815082592931898E-19, -0.9999939076577903929, -0.003490651415223739937 ) ) ;
#73944=ORIENTED_EDGE ( 'NONE', *, *, #113078, .T. ) ;
#73945=ORIENTED_EDGE ( 'NONE', *, *, #44379, .F. ) ;
#73946=EDGE_LOOP ( 'NONE', ( #5350, #22789 ) ) ;
#73947=EDGE_CURVE ( 'NONE', #101350, #90163, #54008, .T. ) ;
#73948=DIRECTION ( 'NONE',  ( 0.000000000000000000, 0.000000000000000000, -1.000000000000000000 ) ) ;
#73949=CONICAL_SURFACE ( 'NONE', #94877, 0.1000000000000000472, 0.003490658503988666988 ) ;
#73951=CARTESIAN_POINT ( 'NONE',  ( -0.4000000000000331624, 12.50000000000000000, -0.7579135962115893799 ) ) ;
#73952=VECTOR ( 'NONE', #2359, 1000.000000000000000 ) ;
#73953=EDGE_CURVE ( 'NONE', #96127, #70629, #68666, .T. ) ;
#73954=DIRECTION ( 'NONE',  ( 0.000000000000000000, 0.000000000000000000, 1.000000000000000000 ) ) ;
#73955=DIRECTION ( 'NONE',  ( 0.000000000000000000, 0.000000000000000000, 1.000000000000000000 ) ) ;
#73957=CARTESIAN_POINT ( 'NONE',  ( 11.84999999999990372, 2.500000000000000000, -6.248780366869526759 ) ) ;
#73958=FACE_OUTER_BOUND ( 'NONE', #16520, .T. ) ;
#73959=CARTESIAN_POINT ( 'NONE',  ( -10.60000000000000320, 2.500000000000000000, -3.983716857408421852 ) ) ;
#73960=AXIS2_PLACEMENT_3D ( 'NONE', #15354, #115490, #104404 ) ;
#73961=FACE_OUTER_BOUND ( 'NONE', #74719, .T. ) ;
#73962=VECTOR ( 'NONE', #4213, 1000.000000000000000 ) ;
#73963=ORIENTED_EDGE ( 'NONE', *, *, #84611, .F. ) ;
#73964=CONICAL_SURFACE ( 'NONE', #109565, 0.1000000000000002554, 0.003490658503988666988 ) ;
#73965=FACE_OUTER_BOUND ( 'NONE', #51441, .T. ) ;
#73966=ORIENTED_EDGE ( 'NONE', *, *, #123275, .T. ) ;
#73967=VERTEX_POINT ( 'NONE', #22898 ) ;
#73968=FACE_OUTER_BOUND ( 'NONE', #65386, .T. ) ;
#73969=DIRECTION ( 'NONE',  ( -0.000000000000000000, -1.000000000000000000, -0.000000000000000000 ) ) ;
#73970=AXIS2_PLACEMENT_3D ( 'NONE', #8866, #29821, #59299 ) ;
#73971=DIRECTION ( 'NONE',  ( -0.000000000000000000, 1.000000000000000000, -0.000000000000000000 ) ) ;
#73972=PLANE ( 'NONE',  #8538 ) ;
#73973=CARTESIAN_POINT ( 'NONE',  ( -4.600000000000024514, 12.50000000000000000, 5.088040615133786027 ) ) ;
#73974=AXIS2_PLACEMENT_3D ( 'NONE', #88511, #128471, #129122 ) ;
#73975=DIRECTION ( 'NONE',  ( -0.000000000000000000, -1.000000000000000000, -0.000000000000000000 ) ) ;
#73976=VECTOR ( 'NONE', #61762, 1000.000000000000000 ) ;
#73977=CIRCLE ( 'NONE', #27911, 0.09999999999999982514 ) ;
#73978=FACE_OUTER_BOUND ( 'NONE', #63389, .T. ) ;
#73979=ORIENTED_EDGE ( 'NONE', *, *, #108801, .T. ) ;
#73980=DIRECTION ( 'NONE',  ( -0.000000000000000000, -1.000000000000000000, -0.000000000000000000 ) ) ;
#73981=AXIS2_PLACEMENT_3D ( 'NONE', #35605, #76814, #4825 ) ;
#73982=AXIS2_PLACEMENT_3D ( 'NONE', #6095, #85941, #125871 ) ;
#73983=CARTESIAN_POINT ( 'NONE',  ( 2.099999999999950351, 2.500000000000000000, -0.1000000000000022815 ) ) ;
#73984=ORIENTED_EDGE ( 'NONE', *, *, #58306, .T. ) ;
#73985=VERTEX_POINT ( 'NONE', #94849 ) ;
#73986=ORIENTED_EDGE ( 'NONE', *, *, #113727, .T. ) ;
#73987=EDGE_CURVE ( 'NONE', #72830, #17629, #70727, .T. ) ;
#73988=ORIENTED_EDGE ( 'NONE', *, *, #40594, .F. ) ;
#73989=LINE ( 'NONE', #113922, #98506 ) ;
#73990=CARTESIAN_POINT ( 'NONE',  ( -11.89999999999999503, 12.50000000000000000, 4.611443907251934426 ) ) ;
#73991=EDGE_CURVE ( 'NONE', #44948, #75085, #81201, .T. ) ;
#73993=CARTESIAN_POINT ( 'NONE',  ( 11.64999999999990443, 12.50000000000000000, -5.802370205355749988 ) ) ;
#73994=EDGE_CURVE ( 'NONE', #117544, #33453, #120890, .T. ) ;
#73995=CARTESIAN_POINT ( 'NONE',  ( 87.50000000000001421, 3.974992050023849810, 6.359987280038159163 ) ) ;
#73997=CARTESIAN_POINT ( 'NONE',  ( -11.89999999999999680, 2.500000000000000000, -3.983716857408423628 ) ) ;
#73998=CIRCLE ( 'NONE', #19619, 0.06509327318403745899 ) ;
#73999=CIRCLE ( 'NONE', #48881, 0.06509327318403745899 ) ;
#74000=LINE ( 'NONE', #15040, #13895 ) ;
#74001=EDGE_CURVE ( 'NONE', #86001, #27095, #3825, .T. ) ;
#74002=CARTESIAN_POINT ( 'NONE',  ( -5.400000000000020783, 2.500000000000000000, 0.7928203230275495672 ) ) ;
#74003=EDGE_LOOP ( 'NONE', ( #75767, #1532 ) ) ;
#74004=CIRCLE ( 'NONE', #92794, 0.09999999999999982514 ) ;
#74005=AXIS2_PLACEMENT_3D ( 'NONE', #3636, #124706, #23261 ) ;
#74007=ORIENTED_EDGE ( 'NONE', *, *, #112691, .T. ) ;
#74008=AXIS2_PLACEMENT_3D ( 'NONE', #82816, #13404, #61232 ) ;
#74010=DIRECTION ( 'NONE',  ( -0.000000000000000000, -1.000000000000000000, -0.000000000000000000 ) ) ;
#74011=LINE ( 'NONE', #13133, #42592 ) ;
#74012=CARTESIAN_POINT ( 'NONE',  ( -6.450000000000017941, 2.500000000000000000, -6.841600689897077814 ) ) ;
#74013=AXIS2_PLACEMENT_3D ( 'NONE', #111173, #32012, #42476 ) ;
#74014=CIRCLE ( 'NONE', #53086, 0.1000000000000002554 ) ;
#74015=VECTOR ( 'NONE', #70835, 1000.000000000000000 ) ;
#74016=AXIS2_PLACEMENT_3D ( 'NONE', #40520, #11015, #31338 ) ;
#74017=ORIENTED_EDGE ( 'NONE', *, *, #119037, .T. ) ;
#74018=DIRECTION ( 'NONE',  ( -0.000000000000000000, -1.000000000000000000, -0.000000000000000000 ) ) ;
#74019=DIRECTION ( 'NONE',  ( -0.000000000000000000, -1.000000000000000000, -0.000000000000000000 ) ) ;
#74020=CARTESIAN_POINT ( 'NONE',  ( -14.99999999999998224, 12.50000000000000000, -0.6928203230275519209 ) ) ;
#74021=EDGE_CURVE ( 'NONE', #54678, #116826, #4496, .T. ) ;
#74022=CARTESIAN_POINT ( 'NONE',  ( 7.299999999999926104, 2.500000000000000000, -3.883716857408426648 ) ) ;
#74023=CARTESIAN_POINT ( 'NONE',  ( 9.149999999999916866, 12.50000000000000000, 7.253104124594885960 ) ) ;
#74024=CIRCLE ( 'NONE', #107474, 0.06509327318403741736 ) ;
#74025=VERTEX_POINT ( 'NONE', #52342 ) ;
#74026=ORIENTED_EDGE ( 'NONE', *, *, #8457, .T. ) ;
#74027=CARTESIAN_POINT ( 'NONE',  ( -6.450000000000019718, 2.500000000000000000, -1.918653347947326004 ) ) ;
#74028=DIRECTION ( 'NONE',  ( 0.000000000000000000, 1.000000000000000000, 0.000000000000000000 ) ) ;
#74029=DIRECTION ( 'NONE',  ( 0.000000000000000000, 0.000000000000000000, -1.000000000000000000 ) ) ;
#74030=VECTOR ( 'NONE', #67854, 1000.000000000000000 ) ;
#74031=DIRECTION ( 'NONE',  ( -0.000000000000000000, -1.000000000000000000, -0.000000000000000000 ) ) ;
#74032=FACE_OUTER_BOUND ( 'NONE', #91957, .T. ) ;
#74033=EDGE_LOOP ( 'NONE', ( #42623, #39106, #64458, #73589 ) ) ;
#74035=ORIENTED_EDGE ( 'NONE', *, *, #25800, .F. ) ;
#74036=CARTESIAN_POINT ( 'NONE',  ( -11.84999999999999787, 2.500000000000000000, -1.718653347947321830 ) ) ;
#74037=CARTESIAN_POINT ( 'NONE',  ( 11.84999999999990727, 12.50000000000000000, 6.148780366869520009 ) ) ;
#74038=DIRECTION ( 'NONE',  ( 0.000000000000000000, -0.000000000000000000, 1.000000000000000000 ) ) ;
#74039=CARTESIAN_POINT ( 'NONE',  ( 3.099999999999945022, 2.500000000000000000, -4.776537180435978414 ) ) ;
#74040=ORIENTED_EDGE ( 'NONE', *, *, #81372, .F. ) ;
#74041=CIRCLE ( 'NONE', #94976, 0.09999999999999999167 ) ;
#74042=CIRCLE ( 'NONE', #94879, 0.06509327318403745899 ) ;
#74043=DIRECTION ( 'NONE',  ( 0.000000000000000000, 0.000000000000000000, -1.000000000000000000 ) ) ;
#74045=VERTEX_POINT ( 'NONE', #93562 ) ;
#74046=DIRECTION ( 'NONE',  ( -0.000000000000000000, -1.000000000000000000, -0.000000000000000000 ) ) ;
#74047=EDGE_CURVE ( 'NONE', #10609, #70290, #47751, .T. ) ;
#74048=ORIENTED_EDGE ( 'NONE', *, *, #128158, .F. ) ;
#74049=CARTESIAN_POINT ( 'NONE',  ( 12.89999999999990088, 2.500000000000000000, -4.330127018922201643 ) ) ;
#74050=CIRCLE ( 'NONE', #42784, 0.06509327318403741736 ) ;
#74051=ORIENTED_EDGE ( 'NONE', *, *, #107820, .F. ) ;
#74052=CARTESIAN_POINT ( 'NONE',  ( -0.8500000000000382805, 2.500000000000000000, -7.188010851410854052 ) ) ;
#74053=DIRECTION ( 'NONE',  ( 0.000000000000000000, 0.000000000000000000, 1.000000000000000000 ) ) ;
#74054=ORIENTED_EDGE ( 'NONE', *, *, #13238, .F. ) ;
#74055=VERTEX_POINT ( 'NONE', #24175 ) ;
#74057=CARTESIAN_POINT ( 'NONE',  ( 4.799999999999937650, 2.500000000000000000, -3.883716857408426648 ) ) ;
#74059=DIRECTION ( 'NONE',  ( 0.000000000000000000, 0.000000000000000000, -1.000000000000000000 ) ) ;
#74060=AXIS2_PLACEMENT_3D ( 'NONE', #114595, #94978, #106080 ) ;
#74061=AXIS2_PLACEMENT_3D ( 'NONE', #99645, #108797, #8023 ) ;
#74062=CARTESIAN_POINT ( 'NONE',  ( 9.599999999999917932, 2.500000000000000000, -0.1000000000000022815 ) ) ;
#74063=CARTESIAN_POINT ( 'NONE',  ( 1.649999999999951505, 2.500000000000000000, -1.572243186433550211 ) ) ;
#74064=DIRECTION ( 'NONE',  ( 0.000000000000000000, 0.000000000000000000, 1.000000000000000000 ) ) ;
#74065=AXIS2_PLACEMENT_3D ( 'NONE', #115250, #25600, #105471 ) ;
#74066=CARTESIAN_POINT ( 'NONE',  ( -5.600000000000020073, 2.500000000000000000, 0.3464101615137736845 ) ) ;
#74067=VECTOR ( 'NONE', #36394, 1000.000000000000000 ) ;
#74068=ORIENTED_EDGE ( 'NONE', *, *, #102902, .F. ) ;
#74069=ADVANCED_FACE ( 'NONE', ( #53636 ), #5865, .T. ) ;
#74070=VERTEX_POINT ( 'NONE', #83741 ) ;
#74071=DIRECTION ( 'NONE',  ( 0.000000000000000000, 0.000000000000000000, -1.000000000000000000 ) ) ;
#74072=DIRECTION ( 'NONE',  ( -0.000000000000000000, 1.000000000000000000, -0.000000000000000000 ) ) ;
#74073=CARTESIAN_POINT ( 'NONE',  ( 7.099999999999926814, 12.50000000000000000, -0.06509327318403970719 ) ) ;
#74074=CARTESIAN_POINT ( 'NONE',  ( 7.099999999999927702, 2.500000000000000000, -3.737306695894649700 ) ) ;
#74075=ORIENTED_EDGE ( 'NONE', *, *, #60271, .T. ) ;
#74076=ORIENTED_EDGE ( 'NONE', *, *, #29472, .T. ) ;
#74077=FACE_BOUND ( 'NONE', #36130, .T. ) ;
#74078=ORIENTED_EDGE ( 'NONE', *, *, #47335, .T. ) ;
#74079=DIRECTION ( 'NONE',  ( -0.000000000000000000, 1.000000000000000000, -0.000000000000000000 ) ) ;
#74080=DIRECTION ( 'NONE',  ( 0.000000000000000000, 0.000000000000000000, 1.000000000000000000 ) ) ;
#74081=ORIENTED_EDGE ( 'NONE', *, *, #65085, .F. ) ;
#74082=DIRECTION ( 'NONE',  ( -0.000000000000000000, -1.000000000000000000, -0.000000000000000000 ) ) ;
#74083=EDGE_CURVE ( 'NONE', #114265, #1501, #64457, .T. ) ;
#74084=DIRECTION ( 'NONE',  ( 0.000000000000000000, -0.9999939076577903929, 0.003490651415223739937 ) ) ;
#74085=CARTESIAN_POINT ( 'NONE',  ( 1.249999999999986899, 12.50000000000000000, 6.495190528383297135 ) ) ;
#74086=CONICAL_SURFACE ( 'NONE', #57359, 0.1000000000000002554, 0.003490658503988666988 ) ;
#74087=DIRECTION ( 'NONE',  ( 0.000000000000000000, 0.000000000000000000, 1.000000000000000000 ) ) ;
#74088=CIRCLE ( 'NONE', #17638, 0.1000000000000002554 ) ;
#74089=DIRECTION ( 'NONE',  ( 0.000000000000000000, 0.000000000000000000, -1.000000000000000000 ) ) ;
#74090=LINE ( 'NONE', #125126, #45331 ) ;
#74091=CIRCLE ( 'NONE', #48967, 0.09999999999999982514 ) ;
#74092=EDGE_CURVE ( 'NONE', #86121, #44827, #85394, .T. ) ;
#74093=CIRCLE ( 'NONE', #34404, 0.09999999999999982514 ) ;
#74094=EDGE_CURVE ( 'NONE', #29442, #44638, #92256, .T. ) ;
#74096=DIRECTION ( 'NONE',  ( -4.274815082592931898E-19, -0.9999939076577903929, -0.003490651415223739937 ) ) ;
#74097=EDGE_CURVE ( 'NONE', #33468, #78082, #72785, .T. ) ;
#74098=ADVANCED_FACE ( 'NONE', ( #3250 ), #74934, .T. ) ;
#74099=CARTESIAN_POINT ( 'NONE',  ( -3.100000000000028955, 2.500000000000000000, 3.983716857408420964 ) ) ;
#74100=EDGE_LOOP ( 'NONE', ( #80798, #32423 ) ) ;
#74102=ORIENTED_EDGE ( 'NONE', *, *, #57071, .T. ) ;
#74103=CONICAL_SURFACE ( 'NONE', #13446, 0.09999999999999999167, 0.003490658503988666988 ) ;
#74104=DIRECTION ( 'NONE',  ( 0.000000000000000000, 0.000000000000000000, 1.000000000000000000 ) ) ;
#74105=EDGE_LOOP ( 'NONE', ( #74547, #6736, #28455, #97750 ) ) ;
#74106=ADVANCED_FACE ( 'NONE', ( #124310 ), #91653, .T. ) ;
#74107=ADVANCED_FACE ( 'NONE', ( #37853 ), #125099, .T. ) ;
#74108=ORIENTED_EDGE ( 'NONE', *, *, #4546, .F. ) ;
#74109=ORIENTED_EDGE ( 'NONE', *, *, #6716, .T. ) ;
#74110=ORIENTED_EDGE ( 'NONE', *, *, #88354, .T. ) ;
#74111=EDGE_CURVE ( 'NONE', #58932, #868, #108376, .T. ) ;
#74112=DIRECTION ( 'NONE',  ( 0.000000000000000000, -0.9999939076577903929, 0.003490651415223739937 ) ) ;
#74113=ADVANCED_FACE ( 'NONE', ( #35923 ), #45694, .T. ) ;
#74114=CIRCLE ( 'NONE', #118004, 0.06509327318403745899 ) ;
#74115=AXIS2_PLACEMENT_3D ( 'NONE', #86282, #24808, #5153 ) ;
#74116=EDGE_CURVE ( 'NONE', #82725, #93012, #62428, .T. ) ;
#74117=CARTESIAN_POINT ( 'NONE',  ( -8.950000000000008171, 2.500000000000000000, 1.818653347947321475 ) ) ;
#74119=CARTESIAN_POINT ( 'NONE',  ( 11.44999999999990514, 12.50000000000000000, 2.446380397790835826 ) ) ;
#74120=DIRECTION ( 'NONE',  ( 0.000000000000000000, 0.000000000000000000, 1.000000000000000000 ) ) ;
#74121=CONICAL_SURFACE ( 'NONE', #21895, 0.09999999999999982514, 0.003490658503988666988 ) ;
#74123=ORIENTED_EDGE ( 'NONE', *, *, #60190, .F. ) ;
#74124=EDGE_CURVE ( 'NONE', #71126, #117070, #118749, .T. ) ;
#74125=DIRECTION ( 'NONE',  ( 0.000000000000000000, 1.000000000000000000, 0.000000000000000000 ) ) ;
#74126=EDGE_LOOP ( 'NONE', ( #19123, #48299, #87638, #95952 ) ) ;
#74127=ORIENTED_EDGE ( 'NONE', *, *, #124345, .F. ) ;
#74128=ORIENTED_EDGE ( 'NONE', *, *, #21327, .F. ) ;
#74129=CARTESIAN_POINT ( 'NONE',  ( -7.050000000000013145, 12.50000000000000000, 2.165063509461097713 ) ) ;
#74130=ORIENTED_EDGE ( 'NONE', *, *, #69967, .T. ) ;
#74131=ORIENTED_EDGE ( 'NONE', *, *, #16426, .F. ) ;
#74132=EDGE_LOOP ( 'NONE', ( #27392, #7650 ) ) ;
#74133=AXIS2_PLACEMENT_3D ( 'NONE', #48884, #60639, #28586 ) ;
#74134=DIRECTION ( 'NONE',  ( 0.000000000000000000, 0.000000000000000000, 1.000000000000000000 ) ) ;
#74135=DIRECTION ( 'NONE',  ( 0.000000000000000000, 0.000000000000000000, 1.000000000000000000 ) ) ;
#74136=DIRECTION ( 'NONE',  ( 0.000000000000000000, 1.000000000000000000, 0.000000000000000000 ) ) ;
#74137=DIRECTION ( 'NONE',  ( 0.000000000000000000, -0.9999939076577903929, 0.003490651415223739937 ) ) ;
#74138=CARTESIAN_POINT ( 'NONE',  ( -3.750000000000031086, 2.500000000000000000, -5.802370205355749988 ) ) ;
#74139=CARTESIAN_POINT ( 'NONE',  ( -5.600000000000020073, 2.500000000000000000, 4.776537180435972196 ) ) ;
#74140=DIRECTION ( 'NONE',  ( -0.000000000000000000, -1.000000000000000000, -0.000000000000000000 ) ) ;
#74141=CONICAL_SURFACE ( 'NONE', #105532, 0.09999999999999982514, 0.003490658503988666988 ) ;
#74142=ORIENTED_EDGE ( 'NONE', *, *, #61719, .F. ) ;
#74143=DIRECTION ( 'NONE',  ( 0.000000000000000000, 0.000000000000000000, 1.000000000000000000 ) ) ;
#74144=VERTEX_POINT ( 'NONE', #65376 ) ;
#74145=CARTESIAN_POINT ( 'NONE',  ( -6.505213034913026604E-15, 2.500000000000000000, 4.330127018922196314 ) ) ;
#74146=VERTEX_POINT ( 'NONE', #16259 ) ;
#74147=EDGE_LOOP ( 'NONE', ( #117244, #74479 ) ) ;
#74148=CARTESIAN_POINT ( 'NONE',  ( -3.750000000000027978, 2.500000000000000000, 7.288010851410849256 ) ) ;
#74150=CIRCLE ( 'NONE', #70039, 0.06509327318403745899 ) ;
#74151=EDGE_CURVE ( 'NONE', #116013, #56139, #62327, .T. ) ;
#74152=CARTESIAN_POINT ( 'NONE',  ( 11.24999999999991118, 12.50000000000000000, -2.922977105672691422 ) ) ;
#74153=CONICAL_SURFACE ( 'NONE', #126664, 0.1000000000000002554, 0.003490658503988666988 ) ;
#74154=ADVANCED_FACE ( 'NONE', ( #16888 ), #56043, .T. ) ;
#74155=ORIENTED_EDGE ( 'NONE', *, *, #48853, .T. ) ;
#74156=CARTESIAN_POINT ( 'NONE',  ( -3.749999999999994671, 2.500000000000000000, -6.495190528383302464 ) ) ;
#74157=ORIENTED_EDGE ( 'NONE', *, *, #66047, .F. ) ;
#74158=DIRECTION ( 'NONE',  ( -4.274815082592931898E-19, -0.9999939076577903929, -0.003490651415223739937 ) ) ;
#74160=DIRECTION ( 'NONE',  ( 0.000000000000000000, 0.000000000000000000, 1.000000000000000000 ) ) ;
#74161=CARTESIAN_POINT ( 'NONE',  ( 7.699999999999925571, 12.50000000000000000, 3.983716857408420076 ) ) ;
#74162=ADVANCED_FACE ( 'NONE', ( #67954 ), #97416, .T. ) ;
#74163=CARTESIAN_POINT ( 'NONE',  ( 7.299999999999924327, 12.50000000000000000, 0.3464101615137735735 ) ) ;
#74164=ORIENTED_EDGE ( 'NONE', *, *, #4353, .T. ) ;
#74165=AXIS2_PLACEMENT_3D ( 'NONE', #82441, #100749, #50378 ) ;
#74166=CIRCLE ( 'NONE', #26041, 0.06509327318403745899 ) ;
#74167=AXIS2_PLACEMENT_3D ( 'NONE', #78607, #38014, #57664 ) ;
#74168=ORIENTED_EDGE ( 'NONE', *, *, #61118, .T. ) ;
#74169=CIRCLE ( 'NONE', #124344, 0.1000000000000000472 ) ;
#74173=LINE ( 'NONE', #45368, #9341 ) ;
#74174=DIRECTION ( 'NONE',  ( 0.000000000000000000, 0.000000000000000000, 1.000000000000000000 ) ) ;
#74175=DIRECTION ( 'NONE',  ( 0.000000000000000000, 0.000000000000000000, 1.000000000000000000 ) ) ;
#74176=LINE ( 'NONE', #46013, #108162 ) ;
#74177=EDGE_LOOP ( 'NONE', ( #65241, #104930 ) ) ;
#74178=DIRECTION ( 'NONE',  ( 0.000000000000000000, 0.000000000000000000, 1.000000000000000000 ) ) ;
#74179=AXIS2_PLACEMENT_3D ( 'NONE', #57567, #26168, #97478 ) ;
#74180=DIRECTION ( 'NONE',  ( 0.000000000000000000, 0.000000000000000000, -1.000000000000000000 ) ) ;
#74181=CARTESIAN_POINT ( 'NONE',  ( -12.49999999999999289, 2.500000000000000000, -0.7928203230275501223 ) ) ;
#74182=CIRCLE ( 'NONE', #30282, 0.06509327318403745899 ) ;
#74183=VERTEX_POINT ( 'NONE', #107240 ) ;
#74184=CIRCLE ( 'NONE', #28215, 0.1000000000000002554 ) ;
#74185=DIRECTION ( 'NONE',  ( 0.000000000000000000, 0.000000000000000000, 1.000000000000000000 ) ) ;
#74186=EDGE_CURVE ( 'NONE', #72457, #128585, #39363, .T. ) ;
#74187=AXIS2_PLACEMENT_3D ( 'NONE', #77651, #118231, #61754 ) ;
#74188=AXIS2_PLACEMENT_3D ( 'NONE', #51718, #5808, #116413 ) ;
#74189=ORIENTED_EDGE ( 'NONE', *, *, #45876, .T. ) ;
#74190=VECTOR ( 'NONE', #112778, 1000.000000000000000 ) ;
#74191=CARTESIAN_POINT ( 'NONE',  ( -8.100000000000013856, 2.500000000000000000, -0.2464101615137782308 ) ) ;
#74192=AXIS2_PLACEMENT_3D ( 'NONE', #46971, #107811, #67200 ) ;
#74193=ORIENTED_EDGE ( 'NONE', *, *, #25003, .F. ) ;
#74194=DIRECTION ( 'NONE',  ( -0.000000000000000000, -1.000000000000000000, -0.000000000000000000 ) ) ;
#74195=PLANE ( 'NONE',  #90566 ) ;
#74196=CARTESIAN_POINT ( 'NONE',  ( 1.649999999999951505, 2.500000000000000000, 1.472243186433545459 ) ) ;
#74197=EDGE_LOOP ( 'NONE', ( #35382, #20532 ) ) ;
#74198=AXIS2_PLACEMENT_3D ( 'NONE', #105852, #34560, #24076 ) ;
#74199=AXIS2_PLACEMENT_3D ( 'NONE', #66340, #57825, #85343 ) ;
#74200=DIRECTION ( 'NONE',  ( -0.000000000000000000, 1.000000000000000000, -0.000000000000000000 ) ) ;
#74201=DIRECTION ( 'NONE',  ( 0.000000000000000000, 0.000000000000000000, 1.000000000000000000 ) ) ;
#74202=AXIS2_PLACEMENT_3D ( 'NONE', #15197, #45990, #114076 ) ;
#74203=ADVANCED_FACE ( 'NONE', ( #126242 ), #116405, .T. ) ;
#74204=EDGE_CURVE ( 'NONE', #112423, #87133, #128184, .T. ) ;
#74205=VERTEX_POINT ( 'NONE', #78453 ) ;
#74206=DIRECTION ( 'NONE',  ( 0.000000000000000000, 1.000000000000000000, 0.000000000000000000 ) ) ;
#74207=ORIENTED_EDGE ( 'NONE', *, *, #41151, .F. ) ;
#74208=EDGE_LOOP ( 'NONE', ( #24946, #68171, #10916, #37396 ) ) ;
#74209=FACE_OUTER_BOUND ( 'NONE', #20991, .T. ) ;
#74210=CARTESIAN_POINT ( 'NONE',  ( 9.349999999999919709, 2.500000000000000000, -6.941600689897078347 ) ) ;
#74211=FACE_OUTER_BOUND ( 'NONE', #121692, .T. ) ;
#74212=EDGE_CURVE ( 'NONE', #86058, #84876, #43557, .T. ) ;
#74213=VERTEX_POINT ( 'NONE', #36595 ) ;
#74214=LINE ( 'NONE', #93852, #124149 ) ;
#74215=CARTESIAN_POINT ( 'NONE',  ( -4.150000000000025224, 2.500000000000000000, -1.472243186433550122 ) ) ;
#74216=AXIS2_PLACEMENT_3D ( 'NONE', #11922, #124467, #51866 ) ;
#74217=EDGE_LOOP ( 'NONE', ( #107600, #56425 ) ) ;
#74218=LINE ( 'NONE', #114140, #119791 ) ;
#74219=DIRECTION ( 'NONE',  ( 0.000000000000000000, -0.9999939076577903929, 0.003490651415223739937 ) ) ;
#74220=CARTESIAN_POINT ( 'NONE',  ( 14.99999999999992895, 2.500000000000000000, -2.276824562219559311E-15 ) ) ;
#74221=CARTESIAN_POINT ( 'NONE',  ( 4.349999999999938360, 2.500000000000000000, 1.818653347947321475 ) ) ;
#74222=CARTESIAN_POINT ( 'NONE',  ( -12.49999999999995914, 2.500000000000000000, -4.330127018922198978 ) ) ;
#74223=LINE ( 'NONE', #125254, #72369 ) ;
#74224=DIRECTION ( 'NONE',  ( -0.000000000000000000, -1.000000000000000000, -0.000000000000000000 ) ) ;
#74225=AXIS2_PLACEMENT_3D ( 'NONE', #29810, #127369, #69731 ) ;
#74226=AXIS2_PLACEMENT_3D ( 'NONE', #39148, #128817, #107853 ) ;
#74227=ORIENTED_EDGE ( 'NONE', *, *, #99876, .T. ) ;
#74228=ORIENTED_EDGE ( 'NONE', *, *, #18874, .T. ) ;
#74229=EDGE_LOOP ( 'NONE', ( #57021, #59987 ) ) ;
#74230=VERTEX_POINT ( 'NONE', #105316 ) ;
#74231=DIRECTION ( 'NONE',  ( -0.000000000000000000, -1.000000000000000000, -0.000000000000000000 ) ) ;
#74232=DIRECTION ( 'NONE',  ( 0.000000000000000000, 1.000000000000000000, 0.000000000000000000 ) ) ;
#74233=DIRECTION ( 'NONE',  ( -4.274815082592931898E-19, -0.9999939076577903929, -0.003490651415223739937 ) ) ;
#74234=VERTEX_POINT ( 'NONE', #15623 ) ;
#74235=FACE_BOUND ( 'NONE', #114935, .T. ) ;
#74236=CARTESIAN_POINT ( 'NONE',  ( -13.09999999999999254, 2.500000000000000000, -0.3464101615137741286 ) ) ;
#74237=CARTESIAN_POINT ( 'NONE',  ( -1.650000000000034772, 2.500000000000000000, 5.802370205355744659 ) ) ;
#74238=AXIS2_PLACEMENT_3D ( 'NONE', #30261, #11226, #19098 ) ;
#74239=FACE_OUTER_BOUND ( 'NONE', #107908, .T. ) ;
#74240=EDGE_CURVE ( 'NONE', #118322, #53342, #76987, .T. ) ;
#74241=CARTESIAN_POINT ( 'NONE',  ( -7.900000000000014566, 2.500000000000000000, -5.022947341949754119 ) ) ;
#74242=AXIS2_PLACEMENT_3D ( 'NONE', #82459, #110605, #20942 ) ;
#74243=DIRECTION ( 'NONE',  ( -0.000000000000000000, -1.000000000000000000, -0.000000000000000000 ) ) ;
#74244=CARTESIAN_POINT ( 'NONE',  ( 12.49999999999990585, 2.500000000000000000, 3.637306695894644726 ) ) ;
#74245=DIRECTION ( 'NONE',  ( 0.000000000000000000, 1.000000000000000000, 0.000000000000000000 ) ) ;
#74246=CARTESIAN_POINT ( 'NONE',  ( 3.149999999999946176, 12.50000000000000000, -6.213873640053564351 ) ) ;
#74247=EDGE_CURVE ( 'NONE', #118333, #7975, #85483, .T. ) ;
#74248=DIRECTION ( 'NONE',  ( 0.000000000000000000, 1.000000000000000000, 0.000000000000000000 ) ) ;
#74249=ADVANCED_FACE ( 'NONE', ( #46375 ), #26752, .T. ) ;
#74250=DIRECTION ( 'NONE',  ( 0.000000000000000000, 0.000000000000000000, 1.000000000000000000 ) ) ;
#74251=CONICAL_SURFACE ( 'NONE', #40919, 0.1000000000000002554, 0.003490658503988666988 ) ;
#74253=EDGE_LOOP ( 'NONE', ( #67974, #104779 ) ) ;
#74255=VERTEX_POINT ( 'NONE', #47046 ) ;
#74256=ORIENTED_EDGE ( 'NONE', *, *, #25155, .F. ) ;
#74257=ADVANCED_FACE ( 'NONE', ( #86955 ), #110526, .T. ) ;
#74258=VERTEX_POINT ( 'NONE', #60731 ) ;
#74259=PLANE ( 'NONE',  #48519 ) ;
#74260=ADVANCED_FACE ( 'NONE', ( #30636 ), #81287, .T. ) ;
#74261=ADVANCED_FACE ( 'NONE', ( #100010 ), #24849, .T. ) ;
#74262=VERTEX_POINT ( 'NONE', #31281 ) ;
#74263=ORIENTED_EDGE ( 'NONE', *, *, #107699, .T. ) ;
#74264=EDGE_CURVE ( 'NONE', #108726, #69317, #16401, .T. ) ;
#74265=FACE_OUTER_BOUND ( 'NONE', #40158, .T. ) ;
#74266=FACE_OUTER_BOUND ( 'NONE', #71675, .T. ) ;
#74267=LINE ( 'NONE', #35008, #124127 ) ;
#74268=LINE ( 'NONE', #12264, #12060 ) ;
#74269=EDGE_CURVE ( 'NONE', #65715, #116743, #51562, .T. ) ;
#74270=AXIS2_PLACEMENT_3D ( 'NONE', #16300, #124989, #85058 ) ;
#74271=ORIENTED_EDGE ( 'NONE', *, *, #77407, .T. ) ;
#74272=DIRECTION ( 'NONE',  ( 0.000000000000000000, -0.000000000000000000, 1.000000000000000000 ) ) ;
#74273=ADVANCED_FACE ( 'NONE', ( #120295 ), #114727, .T. ) ;
#74274=VERTEX_POINT ( 'NONE', #91468 ) ;
#74275=CONICAL_SURFACE ( 'NONE', #84727, 0.1000000000000002554, 0.003490658503988666988 ) ;
#74276=ORIENTED_EDGE ( 'NONE', *, *, #76607, .T. ) ;
#74277=DIRECTION ( 'NONE',  ( -0.000000000000000000, -1.000000000000000000, -0.000000000000000000 ) ) ;
#74278=EDGE_LOOP ( 'NONE', ( #22860, #58193, #122706, #21209 ) ) ;
#74279=AXIS2_PLACEMENT_3D ( 'NONE', #55321, #25857, #96501 ) ;
#74280=CIRCLE ( 'NONE', #34586, 0.06509327318403745899 ) ;
#74281=FACE_OUTER_BOUND ( 'NONE', #58590, .T. ) ;
#74283=VERTEX_POINT ( 'NONE', #108533 ) ;
#74284=DIRECTION ( 'NONE',  ( 0.000000000000000000, -0.9999939076577903929, 0.003490651415223739937 ) ) ;
#74285=CONICAL_SURFACE ( 'NONE', #122405, 0.1000000000000002554, 0.003490658503988666988 ) ;
#74286=CONICAL_SURFACE ( 'NONE', #55499, 0.1000000000000000056, 0.003490658503988666988 ) ;
#74288=CARTESIAN_POINT ( 'NONE',  ( -6.650000000000018119, 2.500000000000000000, -6.395190528383301931 ) ) ;
#74289=CARTESIAN_POINT ( 'NONE',  ( 11.24999999999994316, 2.500000000000000000, 2.265063509461097357 ) ) ;
#74290=FACE_OUTER_BOUND ( 'NONE', #50434, .T. ) ;
#74291=CIRCLE ( 'NONE', #91009, 0.06509327318403745899 ) ;
#74292=CARTESIAN_POINT ( 'NONE',  ( 11.84999999999990727, 12.50000000000000000, 6.148780366869520009 ) ) ;
#74293=ORIENTED_EDGE ( 'NONE', *, *, #99656, .F. ) ;
#74294=DIRECTION ( 'NONE',  ( 0.000000000000000000, 0.000000000000000000, 1.000000000000000000 ) ) ;
#74295=AXIS2_PLACEMENT_3D ( 'NONE', #94577, #23929, #42945 ) ;
#74296=AXIS2_PLACEMENT_3D ( 'NONE', #83890, #61703, #62342 ) ;
#74297=ORIENTED_EDGE ( 'NONE', *, *, #12576, .F. ) ;
#74298=CARTESIAN_POINT ( 'NONE',  ( 87.50000000000002842, 7.032605354647521345, -2.693424153406288379 ) ) ;
#74299=EDGE_LOOP ( 'NONE', ( #41390, #61757 ) ) ;
#74300=FACE_OUTER_BOUND ( 'NONE', #2100, .T. ) ;
#74301=DIRECTION ( 'NONE',  ( 0.000000000000000000, 0.000000000000000000, 1.000000000000000000 ) ) ;
#74302=VECTOR ( 'NONE', #38095, 1000.000000000000000 ) ;
#74303=DIRECTION ( 'NONE',  ( 0.000000000000000000, 1.000000000000000000, 0.000000000000000000 ) ) ;
#74304=FACE_OUTER_BOUND ( 'NONE', #110839, .T. ) ;
#74305=ORIENTED_EDGE ( 'NONE', *, *, #16438, .T. ) ;
#74306=DIRECTION ( 'NONE',  ( 0.000000000000000000, 1.000000000000000000, 0.000000000000000000 ) ) ;
#74307=ADVANCED_FACE ( 'NONE', ( #90826 ), #41107, .T. ) ;
#74308=DIRECTION ( 'NONE',  ( -0.000000000000000000, 1.000000000000000000, -0.000000000000000000 ) ) ;
#74309=ADVANCED_FACE ( 'NONE', ( #80378 ), #111084, .T. ) ;
#74310=ORIENTED_EDGE ( 'NONE', *, *, #84906, .F. ) ;
#74311=ORIENTED_EDGE ( 'NONE', *, *, #122403, .F. ) ;
#74312=VERTEX_POINT ( 'NONE', #61377 ) ;
#74313=CARTESIAN_POINT ( 'NONE',  ( -1.050000000000038680, 2.500000000000000000, 2.511473670974873507 ) ) ;
#74314=FACE_OUTER_BOUND ( 'NONE', #125698, .T. ) ;
#74316=AXIS2_PLACEMENT_3D ( 'NONE', #58316, #89691, #10476 ) ;
#74317=FACE_OUTER_BOUND ( 'NONE', #69885, .T. ) ;
#74318=CARTESIAN_POINT ( 'NONE',  ( 17.49862860983167323, 2.500000000000000000, -4.081131818001370704 ) ) ;
#74319=DIRECTION ( 'NONE',  ( 0.000000000000000000, -0.9999939076577903929, 0.003490651415223739937 ) ) ;
#74320=VERTEX_POINT ( 'NONE', #20156 ) ;
#74321=AXIS2_PLACEMENT_3D ( 'NONE', #41710, #33181, #43014 ) ;
#74322=DIRECTION ( 'NONE',  ( -0.000000000000000000, 1.000000000000000000, -0.000000000000000000 ) ) ;
#74323=EDGE_LOOP ( 'NONE', ( #12032, #112967 ) ) ;
#74324=DIRECTION ( 'NONE',  ( 0.000000000000000000, -0.000000000000000000, 1.000000000000000000 ) ) ;
#74325=CARTESIAN_POINT ( 'NONE',  ( -8.300000000000011369, 2.500000000000000000, -0.1000000000000022815 ) ) ;
#74326=LINE ( 'NONE', #3014, #89808 ) ;
#74327=ORIENTED_EDGE ( 'NONE', *, *, #103913, .F. ) ;
#74328=CIRCLE ( 'NONE', #47246, 0.06509327318403745899 ) ;
#74329=VECTOR ( 'NONE', #70525, 1000.000000000000000 ) ;
#74330=DIRECTION ( 'NONE',  ( -0.000000000000000000, 1.000000000000000000, -0.000000000000000000 ) ) ;
#74331=LINE ( 'NONE', #103791, #92282 ) ;
#74332=ORIENTED_EDGE ( 'NONE', *, *, #88023, .T. ) ;
#74333=FACE_OUTER_BOUND ( 'NONE', #90030, .T. ) ;
#74334=ADVANCED_FACE ( 'NONE', ( #48990 ), #93812, .T. ) ;
#74335=CIRCLE ( 'NONE', #11643, 0.06509327318403745899 ) ;
#74336=VECTOR ( 'NONE', #38860, 1000.000000000000000 ) ;
#74337=VERTEX_POINT ( 'NONE', #9689 ) ;
#74338=VERTEX_POINT ( 'NONE', #101303 ) ;
#74339=LINE ( 'NONE', #53422, #123980 ) ;
#74340=EDGE_LOOP ( 'NONE', ( #10285, #67930, #43939, #25351 ) ) ;
#74341=CARTESIAN_POINT ( 'NONE',  ( 17.17161331427240256, 0.4678040054248072122, -5.513957101008877260 ) ) ;
#74342=CARTESIAN_POINT ( 'NONE',  ( 10.19999999999991580, 2.500000000000000000, -0.2464101615137783419 ) ) ;
#74343=DIRECTION ( 'NONE',  ( -0.000000000000000000, -1.000000000000000000, -0.000000000000000000 ) ) ;
#74344=EDGE_CURVE ( 'NONE', #31556, #47635, #106325, .T. ) ;
#74345=ORIENTED_EDGE ( 'NONE', *, *, #69687, .F. ) ;
#74346=DIRECTION ( 'NONE',  ( 0.000000000000000000, 0.000000000000000000, 1.000000000000000000 ) ) ;
#74347=FACE_OUTER_BOUND ( 'NONE', #103300, .T. ) ;
#74348=ORIENTED_EDGE ( 'NONE', *, *, #1078, .F. ) ;
#74349=EDGE_CURVE ( 'NONE', #77555, #47068, #75024, .T. ) ;
#74350=CARTESIAN_POINT ( 'NONE',  ( 9.599999999999917932, 2.500000000000000000, -0.7928203230275542301 ) ) ;
#74351=CARTESIAN_POINT ( 'NONE',  ( -10.65000000000000213, 2.500000000000000000, 6.148780366869520009 ) ) ;
#74352=EDGE_CURVE ( 'NONE', #17807, #29513, #18589, .T. ) ;
#74353=CIRCLE ( 'NONE', #91076, 0.1000000000000000472 ) ;
#74354=VERTEX_POINT ( 'NONE', #128850 ) ;
#74355=AXIS2_PLACEMENT_3D ( 'NONE', #28372, #87901, #95811 ) ;
#74356=ORIENTED_EDGE ( 'NONE', *, *, #79204, .T. ) ;
#74357=ADVANCED_FACE ( 'NONE', ( #39179 ), #37379, .T. ) ;
#74358=VECTOR ( 'NONE', #31655, 1000.000000000000000 ) ;
#74359=EDGE_LOOP ( 'NONE', ( #61564, #67470, #51082, #71129 ) ) ;
#74360=CARTESIAN_POINT ( 'NONE',  ( -5.850000000000022737, 2.500000000000000000, -6.395190528383301931 ) ) ;
#74361=DIRECTION ( 'NONE',  ( 0.000000000000000000, -0.9999939076577903929, 0.003490651415223739937 ) ) ;
#74362=DIRECTION ( 'NONE',  ( 0.000000000000000000, 0.000000000000000000, 1.000000000000000000 ) ) ;
#74363=EDGE_CURVE ( 'NONE', #88700, #1645, #69236, .T. ) ;
#74364=FACE_BOUND ( 'NONE', #36712, .T. ) ;
#74367=CARTESIAN_POINT ( 'NONE',  ( 14.39999999999989555, 2.500000000000000000, 0.3464101615137736845 ) ) ;
#74368=DIRECTION ( 'NONE',  ( 0.000000000000000000, 1.000000000000000000, 0.000000000000000000 ) ) ;
#74369=CARTESIAN_POINT ( 'NONE',  ( 8.299999999999922551, 12.50000000000000000, 4.330127018922196314 ) ) ;
#74370=LINE ( 'NONE', #4309, #33923 ) ;
#74371=AXIS2_PLACEMENT_3D ( 'NONE', #118112, #96521, #67055 ) ;
#74372=CARTESIAN_POINT ( 'NONE',  ( -11.05000000000000249, 12.50000000000000000, -1.818653347947322141 ) ) ;
#74373=FACE_OUTER_BOUND ( 'NONE', #68026, .T. ) ;
#74374=CIRCLE ( 'NONE', #107823, 0.06509327318403745899 ) ;
#74375=CONICAL_SURFACE ( 'NONE', #5414, 0.1000000000000002554, 0.003490658503988666988 ) ;
#74377=AXIS2_PLACEMENT_3D ( 'NONE', #122573, #34850, #85211 ) ;
#74378=VERTEX_POINT ( 'NONE', #129494 ) ;
#74379=VERTEX_POINT ( 'NONE', #39815 ) ;
#74380=EDGE_LOOP ( 'NONE', ( #79563, #128676, #47985, #59923 ) ) ;
#74381=ORIENTED_EDGE ( 'NONE', *, *, #95970, .F. ) ;
#74382=AXIS2_PLACEMENT_3D ( 'NONE', #54349, #93638, #35368 ) ;
#74383=ORIENTED_EDGE ( 'NONE', *, *, #85649, .T. ) ;
#74384=DIRECTION ( 'NONE',  ( 0.000000000000000000, 0.000000000000000000, 1.000000000000000000 ) ) ;
#74385=DIRECTION ( 'NONE',  ( -0.000000000000000000, 1.000000000000000000, -0.000000000000000000 ) ) ;
#74386=ORIENTED_EDGE ( 'NONE', *, *, #32744, .F. ) ;
#74387=FACE_BOUND ( 'NONE', #32969, .T. ) ;
#74388=PLANE ( 'NONE',  #83384 ) ;
#74389=EDGE_CURVE ( 'NONE', #79739, #11888, #29988, .T. ) ;
#74390=CARTESIAN_POINT ( 'NONE',  ( -3.300000000000027800, 2.500000000000000000, -4.330127018922201643 ) ) ;
#74391=EDGE_LOOP ( 'NONE', ( #48820, #103940, #88837, #88880 ) ) ;
#74392=DIRECTION ( 'NONE',  ( 0.000000000000000000, 0.000000000000000000, -1.000000000000000000 ) ) ;
#74393=DIRECTION ( 'NONE',  ( 0.000000000000000000, 0.000000000000000000, 1.000000000000000000 ) ) ;
#74394=EDGE_CURVE ( 'NONE', #38823, #129286, #123055, .T. ) ;
#74395=CARTESIAN_POINT ( 'NONE',  ( -6.650000000000015454, 12.50000000000000000, 2.792790559304612064 ) ) ;
#74396=AXIS2_PLACEMENT_3D ( 'NONE', #64735, #105958, #66661 ) ;
#74397=ORIENTED_EDGE ( 'NONE', *, *, #69783, .F. ) ;
#74398=CARTESIAN_POINT ( 'NONE',  ( 2.699999999999947331, 2.500000000000000000, -4.676537180435978769 ) ) ;
#74399=EDGE_CURVE ( 'NONE', #77648, #109309, #66605, .T. ) ;
#74400=VERTEX_POINT ( 'NONE', #25791 ) ;
#74401=ORIENTED_EDGE ( 'NONE', *, *, #97756, .T. ) ;
#74402=ORIENTED_EDGE ( 'NONE', *, *, #116074, .T. ) ;
#74403=EDGE_CURVE ( 'NONE', #9181, #111170, #10187, .T. ) ;
#74404=CARTESIAN_POINT ( 'NONE',  ( -5.650000000000019895, 2.500000000000000000, 6.841600689897072485 ) ) ;
#74405=CARTESIAN_POINT ( 'NONE',  ( -7.700000000000016165, 2.500000000000000000, -3.983716857408426293 ) ) ;
#74406=AXIS2_PLACEMENT_3D ( 'NONE', #52346, #12414, #72003 ) ;
#74407=DIRECTION ( 'NONE',  ( 0.000000000000000000, 0.000000000000000000, -1.000000000000000000 ) ) ;
#74408=EDGE_CURVE ( 'NONE', #97087, #112557, #83354, .T. ) ;
#74409=ORIENTED_EDGE ( 'NONE', *, *, #121385, .F. ) ;
#74410=FACE_OUTER_BOUND ( 'NONE', #91981, .T. ) ;
#74411=AXIS2_PLACEMENT_3D ( 'NONE', #62323, #91126, #2731 ) ;
#74412=EDGE_CURVE ( 'NONE', #31054, #37520, #26902, .T. ) ;
#74413=AXIS2_PLACEMENT_3D ( 'NONE', #50713, #2240, #31722 ) ;
#74415=AXIS2_PLACEMENT_3D ( 'NONE', #60856, #60236, #50387 ) ;
#74416=CARTESIAN_POINT ( 'NONE',  ( -7.950000000000012612, 12.50000000000000000, -2.165063509461101710 ) ) ;
#74417=EDGE_CURVE ( 'NONE', #61868, #105096, #54591, .T. ) ;
#74419=DIRECTION ( 'NONE',  ( 0.000000000000000000, 0.000000000000000000, -1.000000000000000000 ) ) ;
#74420=EDGE_LOOP ( 'NONE', ( #25213, #203, #33361, #32402 ) ) ;
#74421=CARTESIAN_POINT ( 'NONE',  ( -13.09999999999999076, 12.50000000000000000, 4.741630453620009789 ) ) ;
#74422=ORIENTED_EDGE ( 'NONE', *, *, #89075, .T. ) ;
#74423=DIRECTION ( 'NONE',  ( 0.000000000000000000, 1.000000000000000000, 0.000000000000000000 ) ) ;
#74424=ADVANCED_FACE ( 'NONE', ( #72491 ), #125201, .T. ) ;
#74425=CIRCLE ( 'NONE', #9667, 0.06509327318403745899 ) ;
#74426=EDGE_CURVE ( 'NONE', #49764, #82278, #52051, .T. ) ;
#74427=VERTEX_POINT ( 'NONE', #52194 ) ;
#74428=AXIS2_PLACEMENT_3D ( 'NONE', #46401, #95520, #56222 ) ;
#74429=CIRCLE ( 'NONE', #43060, 0.06509327318403745899 ) ;
#74430=ORIENTED_EDGE ( 'NONE', *, *, #25474, .F. ) ;
#74431=DIRECTION ( 'NONE',  ( 0.000000000000000000, 0.000000000000000000, 1.000000000000000000 ) ) ;
#74432=CARTESIAN_POINT ( 'NONE',  ( -1.850000000000033396, 2.500000000000000000, -1.818653347947325916 ) ) ;
#74433=CARTESIAN_POINT ( 'NONE',  ( 8.749999999999918288, 12.50000000000000000, -1.472243186433550122 ) ) ;
#74434=DIRECTION ( 'NONE',  ( 0.000000000000000000, 0.000000000000000000, -1.000000000000000000 ) ) ;
#74435=CARTESIAN_POINT ( 'NONE',  ( 3.949999999999942446, 12.50000000000000000, -2.511473670974877948 ) ) ;
#74436=ORIENTED_EDGE ( 'NONE', *, *, #9685, .F. ) ;
#74437=ORIENTED_EDGE ( 'NONE', *, *, #98624, .F. ) ;
#74438=PLANE ( 'NONE',  #64316 ) ;
#74439=CONICAL_SURFACE ( 'NONE', #63972, 0.1000000000000002554, 0.003490658503988666988 ) ;
#74440=DIRECTION ( 'NONE',  ( -0.000000000000000000, 1.000000000000000000, -0.000000000000000000 ) ) ;
#74441=CARTESIAN_POINT ( 'NONE',  ( -4.350000000000023626, 2.500000000000000000, -1.818653347947325916 ) ) ;
#74443=VERTEX_POINT ( 'NONE', #104979 ) ;
#74444=LINE ( 'NONE', #84245, #97972 ) ;
#74445=ORIENTED_EDGE ( 'NONE', *, *, #104266, .T. ) ;
#74446=DIRECTION ( 'NONE',  ( -0.000000000000000000, 1.000000000000000000, -0.000000000000000000 ) ) ;
#74447=DIRECTION ( 'NONE',  ( 0.000000000000000000, 0.000000000000000000, 1.000000000000000000 ) ) ;
#74448=VERTEX_POINT ( 'NONE', #124647 ) ;
#74449=DIRECTION ( 'NONE',  ( 0.000000000000000000, 1.000000000000000000, 0.000000000000000000 ) ) ;
#74450=FACE_OUTER_BOUND ( 'NONE', #124501, .T. ) ;
#74451=PLANE ( 'NONE',  #107444 ) ;
#74452=CARTESIAN_POINT ( 'NONE',  ( 5.849999999999933920, 2.500000000000000000, -2.065063509461102065 ) ) ;
#74453=ORIENTED_EDGE ( 'NONE', *, *, #104692, .F. ) ;
#74454=FACE_OUTER_BOUND ( 'NONE', #102672, .T. ) ;
#74455=CIRCLE ( 'NONE', #55663, 0.1000000000000002554 ) ;
#74456=ADVANCED_FACE ( 'NONE', ( #46087 ), #102219, .T. ) ;
#74457=AXIS2_PLACEMENT_3D ( 'NONE', #116648, #88470, #40038 ) ;
#74458=CARTESIAN_POINT ( 'NONE',  ( 87.50000000000001421, -3.974992050023847145, 6.359987280038161828 ) ) ;
#74459=VERTEX_POINT ( 'NONE', #45450 ) ;
#74460=ORIENTED_EDGE ( 'NONE', *, *, #28598, .F. ) ;
#74462=DIRECTION ( 'NONE',  ( -0.000000000000000000, 1.000000000000000000, -0.000000000000000000 ) ) ;
#74463=LINE ( 'NONE', #122927, #104308 ) ;
#74464=FACE_OUTER_BOUND ( 'NONE', #4225, .T. ) ;
#74465=VECTOR ( 'NONE', #65781, 1000.000000000000000 ) ;
#74466=CARTESIAN_POINT ( 'NONE',  ( -1.850000000000033396, 2.500000000000000000, -6.048780366869526581 ) ) ;
#74467=AXIS2_PLACEMENT_3D ( 'NONE', #94011, #25254, #72451 ) ;
#74468=EDGE_CURVE ( 'NONE', #77466, #87148, #62523, .T. ) ;
#74469=CARTESIAN_POINT ( 'NONE',  ( 11.04999999999991012, 12.50000000000000000, -1.818653347947326138 ) ) ;
#74470=CARTESIAN_POINT ( 'NONE',  ( 9.799999999999917222, 2.500000000000000000, 0.4464101615137735513 ) ) ;
#74471=CARTESIAN_POINT ( 'NONE',  ( 13.54999999999989946, 2.500000000000000000, 2.511473670974873507 ) ) ;
#74472=DIRECTION ( 'NONE',  ( 0.000000000000000000, 1.000000000000000000, 0.000000000000000000 ) ) ;
#74474=AXIS2_PLACEMENT_3D ( 'NONE', #127134, #78013, #27606 ) ;
#74475=CONICAL_SURFACE ( 'NONE', #24393, 0.1000000000000000472, 0.003490658503988666988 ) ;
#74476=VERTEX_POINT ( 'NONE', #76190 ) ;
#74477=ORIENTED_EDGE ( 'NONE', *, *, #104508, .T. ) ;
#74478=VECTOR ( 'NONE', #110023, 1000.000000000000000 ) ;
#74479=ORIENTED_EDGE ( 'NONE', *, *, #37984, .F. ) ;
#74480=ORIENTED_EDGE ( 'NONE', *, *, #47656, .T. ) ;
#74481=LINE ( 'NONE', #99601, #81290 ) ;
#74482=DIRECTION ( 'NONE',  ( -0.000000000000000000, 1.000000000000000000, -0.000000000000000000 ) ) ;
#74483=CARTESIAN_POINT ( 'NONE',  ( 8.349999999999919709, 2.500000000000000000, -2.957883832488653830 ) ) ;
#74484=ORIENTED_EDGE ( 'NONE', *, *, #76192, .F. ) ;
#74485=CARTESIAN_POINT ( 'NONE',  ( 20.59313469514024320, -2.666874593322334785, -2.243770147468747034 ) ) ;
#74486=PLANE ( 'NONE',  #34502 ) ;
#74487=DIRECTION ( 'NONE',  ( -0.000000000000000000, 1.000000000000000000, -0.000000000000000000 ) ) ;
#74488=VERTEX_POINT ( 'NONE', #92105 ) ;
#74489=DIRECTION ( 'NONE',  ( 0.000000000000000000, 1.000000000000000000, 0.000000000000000000 ) ) ;
#74490=AXIS2_PLACEMENT_3D ( 'NONE', #119630, #48326, #48992 ) ;
#74491=DIRECTION ( 'NONE',  ( 0.000000000000000000, 0.000000000000000000, 1.000000000000000000 ) ) ;
#74492=ORIENTED_EDGE ( 'NONE', *, *, #90635, .F. ) ;
#74493=CIRCLE ( 'NONE', #114208, 0.09999999999999982514 ) ;
#74494=ORIENTED_EDGE ( 'NONE', *, *, #114636, .T. ) ;
#74495=ORIENTED_EDGE ( 'NONE', *, *, #49900, .T. ) ;
#74496=ORIENTED_EDGE ( 'NONE', *, *, #42842, .T. ) ;
#74498=AXIS2_PLACEMENT_3D ( 'NONE', #77147, #88220, #6432 ) ;
#74499=DIRECTION ( 'NONE',  ( 0.000000000000000000, 1.000000000000000000, 0.000000000000000000 ) ) ;
#74500=DIRECTION ( 'NONE',  ( 0.000000000000000000, 0.000000000000000000, 1.000000000000000000 ) ) ;
#74501=AXIS2_PLACEMENT_3D ( 'NONE', #99017, #29627, #68903 ) ;
#74502=CARTESIAN_POINT ( 'NONE',  ( -7.950000000000012612, 2.500000000000000000, -2.165063509461101710 ) ) ;
#74503=EDGE_CURVE ( 'NONE', #47024, #103084, #77080, .T. ) ;
#74504=VERTEX_POINT ( 'NONE', #66357 ) ;
#74505=LINE ( 'NONE', #73856, #23052 ) ;
#74506=EDGE_LOOP ( 'NONE', ( #101342, #69019, #26092, #70635 ) ) ;
#74507=CARTESIAN_POINT ( 'NONE',  ( 13.09999999999990195, 12.50000000000000000, -3.983716857408426293 ) ) ;
#74508=CARTESIAN_POINT ( 'NONE',  ( 4.848431875658358869, -2.500000000000000000, -8.943854603575022821 ) ) ;
#74509=EDGE_CURVE ( 'NONE', #121191, #4941, #79155, .T. ) ;
#74510=ADVANCED_FACE ( 'NONE', ( #112410 ), #31915, .T. ) ;
#74512=CARTESIAN_POINT ( 'NONE',  ( -11.64999999999999680, 2.500000000000000000, -6.395190528383298378 ) ) ;
#74513=ADVANCED_FACE ( 'NONE', ( #44805 ), #129337, .T. ) ;
#74514=VECTOR ( 'NONE', #46044, 1000.000000000000000 ) ;
#74515=ORIENTED_EDGE ( 'NONE', *, *, #61960, .T. ) ;
#74516=CIRCLE ( 'NONE', #20138, 0.06509327318403745899 ) ;
#74517=AXIS2_PLACEMENT_3D ( 'NONE', #90321, #9204, #19677 ) ;
#74518=ORIENTED_EDGE ( 'NONE', *, *, #48102, .F. ) ;
#74519=EDGE_CURVE ( 'NONE', #121477, #59645, #56135, .T. ) ;
#74520=EDGE_CURVE ( 'NONE', #17094, #83056, #33281, .T. ) ;
#74521=VERTEX_POINT ( 'NONE', #25141 ) ;
#74522=DIRECTION ( 'NONE',  ( 0.000000000000000000, 1.000000000000000000, 0.000000000000000000 ) ) ;
#74523=DIRECTION ( 'NONE',  ( 0.000000000000000000, 0.000000000000000000, -1.000000000000000000 ) ) ;
#74524=DIRECTION ( 'NONE',  ( -4.274815082592931898E-19, -0.9999939076577903929, -0.003490651415223739937 ) ) ;
#74525=EDGE_CURVE ( 'NONE', #84079, #36965, #99704, .T. ) ;
#74526=FACE_BOUND ( 'NONE', #11866, .T. ) ;
#74527=DIRECTION ( 'NONE',  ( 0.000000000000000000, 0.000000000000000000, 1.000000000000000000 ) ) ;
#74528=DIRECTION ( 'NONE',  ( 0.000000000000000000, 1.000000000000000000, 0.000000000000000000 ) ) ;
#74529=FACE_OUTER_BOUND ( 'NONE', #108059, .T. ) ;
#74531=FACE_OUTER_BOUND ( 'NONE', #115041, .T. ) ;
#74532=PLANE ( 'NONE',  #970 ) ;
#74533=ORIENTED_EDGE ( 'NONE', *, *, #65088, .F. ) ;
#74534=CARTESIAN_POINT ( 'NONE',  ( -8.749999999999976907, 2.500000000000000000, -6.395190528383296602 ) ) ;
#74535=EDGE_LOOP ( 'NONE', ( #40219, #121672, #66225, #92448 ) ) ;
#74536=ORIENTED_EDGE ( 'NONE', *, *, #114133, .T. ) ;
#74537=ORIENTED_EDGE ( 'NONE', *, *, #61570, .T. ) ;
#74538=ORIENTED_EDGE ( 'NONE', *, *, #42776, .F. ) ;
#74539=CARTESIAN_POINT ( 'NONE',  ( 12.29999999999990656, 12.50000000000000000, 3.983716857408420964 ) ) ;
#74540=FACE_BOUND ( 'NONE', #80643, .T. ) ;
#74541=FACE_OUTER_BOUND ( 'NONE', #73596, .T. ) ;
#74542=CIRCLE ( 'NONE', #76596, 0.09999999999999999167 ) ;
#74543=AXIS2_PLACEMENT_3D ( 'NONE', #47769, #46457, #17642 ) ;
#74544=ORIENTED_EDGE ( 'NONE', *, *, #69026, .T. ) ;
#74545=CARTESIAN_POINT ( 'NONE',  ( 14.34999999999989306, 2.500000000000000000, -1.818653347947326138 ) ) ;
#74546=DIRECTION ( 'NONE',  ( 0.000000000000000000, -0.000000000000000000, 1.000000000000000000 ) ) ;
#74547=ORIENTED_EDGE ( 'NONE', *, *, #91670, .F. ) ;
#74548=DIRECTION ( 'NONE',  ( -0.000000000000000000, 1.000000000000000000, -0.000000000000000000 ) ) ;
#74549=DIRECTION ( 'NONE',  ( 0.000000000000000000, -0.000000000000000000, 1.000000000000000000 ) ) ;
#74550=CIRCLE ( 'NONE', #120528, 0.06509327318403745899 ) ;
#74551=ADVANCED_FACE ( 'NONE', ( #68286 ), #59801, .T. ) ;
#74552=ORIENTED_EDGE ( 'NONE', *, *, #15215, .F. ) ;
#74553=EDGE_CURVE ( 'NONE', #47322, #10760, #104081, .T. ) ;
#74554=CARTESIAN_POINT ( 'NONE',  ( -5.850000000000019185, 12.50000000000000000, 6.560283801567334372 ) ) ;
#74555=CARTESIAN_POINT ( 'NONE',  ( -7.050000000000013145, 12.50000000000000000, 6.430097255199259010 ) ) ;
#74556=EDGE_CURVE ( 'NONE', #72795, #46368, #47374, .T. ) ;
#74557=AXIS2_PLACEMENT_3D ( 'NONE', #87177, #89767, #61615 ) ;
#74558=AXIS2_PLACEMENT_3D ( 'NONE', #29461, #69365, #37354 ) ;
#74559=ORIENTED_EDGE ( 'NONE', *, *, #56081, .T. ) ;
#74560=CIRCLE ( 'NONE', #116312, 0.06509327318403745899 ) ;
#74562=CARTESIAN_POINT ( 'NONE',  ( 13.09999999999990195, 2.500000000000000000, 3.983716857408420076 ) ) ;
#74563=LINE ( 'NONE', #114481, #118309 ) ;
#74564=ADVANCED_FACE ( 'NONE', ( #38876 ), #9987, .T. ) ;
#74565=EDGE_CURVE ( 'NONE', #21407, #71164, #97813, .T. ) ;
#74566=ORIENTED_EDGE ( 'NONE', *, *, #78991, .T. ) ;
#74567=ORIENTED_EDGE ( 'NONE', *, *, #85001, .T. ) ;
#74568=FACE_OUTER_BOUND ( 'NONE', #103779, .T. ) ;
#74569=VERTEX_POINT ( 'NONE', #77469 ) ;
#74570=CARTESIAN_POINT ( 'NONE',  ( -2.500000000000031086, 12.50000000000000000, 3.637306695894644726 ) ) ;
#74571=CARTESIAN_POINT ( 'NONE',  ( -8.300000000000011369, 2.500000000000000000, -4.330127018922201643 ) ) ;
#74572=ADVANCED_FACE ( 'NONE', ( #87281 ), #27006, .T. ) ;
#74573=ADVANCED_FACE ( 'NONE', ( #29664 ), #59136, .T. ) ;
#74574=ORIENTED_EDGE ( 'NONE', *, *, #5676, .F. ) ;
#74575=DIRECTION ( 'NONE',  ( 0.000000000000000000, 0.000000000000000000, 1.000000000000000000 ) ) ;
#74576=DIRECTION ( 'NONE',  ( 0.000000000000000000, 0.000000000000000000, -1.000000000000000000 ) ) ;
#74577=DIRECTION ( 'NONE',  ( 0.000000000000000000, 1.000000000000000000, 0.000000000000000000 ) ) ;
#74578=CARTESIAN_POINT ( 'NONE',  ( 0.3999999999999568345, 12.50000000000000000, -5.022947341949754119 ) ) ;
#74579=AXIS2_PLACEMENT_3D ( 'NONE', #74416, #35778, #76354 ) ;
#74580=DIRECTION ( 'NONE',  ( 0.000000000000000000, 0.000000000000000000, 1.000000000000000000 ) ) ;
#74581=EDGE_CURVE ( 'NONE', #51138, #69316, #89687, .T. ) ;
#74582=AXIS2_PLACEMENT_3D ( 'NONE', #17221, #15299, #106911 ) ;
#74583=EDGE_LOOP ( 'NONE', ( #96358, #103852 ) ) ;
#74584=ORIENTED_EDGE ( 'NONE', *, *, #9143, .F. ) ;
#74585=LINE ( 'NONE', #79113, #47513 ) ;
#74586=CIRCLE ( 'NONE', #34901, 0.1000000000000002554 ) ;
#74588=DIRECTION ( 'NONE',  ( -0.000000000000000000, 1.000000000000000000, -0.000000000000000000 ) ) ;
#74589=EDGE_LOOP ( 'NONE', ( #124844, #29612, #108972, #113451 ) ) ;
#74590=EDGE_LOOP ( 'NONE', ( #113617, #8943, #47077, #90770 ) ) ;
#74591=ORIENTED_EDGE ( 'NONE', *, *, #16369, .F. ) ;
#74592=DIRECTION ( 'NONE',  ( 0.000000000000000000, 0.000000000000000000, 1.000000000000000000 ) ) ;
#74593=CONICAL_SURFACE ( 'NONE', #99737, 0.1000000000000000056, 0.003490658503988666988 ) ;
#74594=FACE_OUTER_BOUND ( 'NONE', #44221, .T. ) ;
#74595=DIRECTION ( 'NONE',  ( 0.000000000000000000, 1.000000000000000000, 0.000000000000000000 ) ) ;
#74596=AXIS2_PLACEMENT_3D ( 'NONE', #40714, #31516, #11219 ) ;
#74598=CARTESIAN_POINT ( 'NONE',  ( 4.349999999999936584, 12.50000000000000000, 6.148780366869520009 ) ) ;
#74599=DIRECTION ( 'NONE',  ( -0.000000000000000000, 1.000000000000000000, -0.000000000000000000 ) ) ;
#74600=DIRECTION ( 'NONE',  ( 0.000000000000000000, 1.000000000000000000, 0.000000000000000000 ) ) ;
#74601=DIRECTION ( 'NONE',  ( 0.000000000000000000, 1.000000000000000000, 0.000000000000000000 ) ) ;
#74602=CARTESIAN_POINT ( 'NONE',  ( 1.049999999999953637, 2.500000000000000000, 2.611473670974873151 ) ) ;
#74603=CONICAL_SURFACE ( 'NONE', #89272, 0.1000000000000002554, 0.003490658503988666988 ) ;
#74604=DIRECTION ( 'NONE',  ( 0.000000000000000000, 0.000000000000000000, -1.000000000000000000 ) ) ;
#74605=AXIS2_PLACEMENT_3D ( 'NONE', #21070, #60998, #91112 ) ;
#74606=ORIENTED_EDGE ( 'NONE', *, *, #86182, .F. ) ;
#74607=CIRCLE ( 'NONE', #11900, 0.1000000000000000472 ) ;
#74608=AXIS2_PLACEMENT_3D ( 'NONE', #76510, #4505, #75214 ) ;
#74609=LINE ( 'NONE', #114517, #31942 ) ;
#74610=ORIENTED_EDGE ( 'NONE', *, *, #24128, .F. ) ;
#74611=EDGE_LOOP ( 'NONE', ( #39746, #118097, #70828, #101157 ) ) ;
#74612=PLANE ( 'NONE',  #81754 ) ;
#74613=DIRECTION ( 'NONE',  ( 0.000000000000000000, 1.000000000000000000, 0.000000000000000000 ) ) ;
#74615=CARTESIAN_POINT ( 'NONE',  ( 3.949999999999941558, 12.50000000000000000, -1.818653347947326138 ) ) ;
#74616=ADVANCED_FACE ( 'NONE', ( #27719 ), #43456, .T. ) ;
#74617=DIRECTION ( 'NONE',  ( -0.000000000000000000, 1.000000000000000000, -0.000000000000000000 ) ) ;
#74618=DIRECTION ( 'NONE',  ( 0.000000000000000000, 0.000000000000000000, -1.000000000000000000 ) ) ;
#74619=DIRECTION ( 'NONE',  ( 0.000000000000000000, 0.000000000000000000, -1.000000000000000000 ) ) ;
#74620=EDGE_LOOP ( 'NONE', ( #12053, #38405, #31470, #13386 ) ) ;
#74621=CARTESIAN_POINT ( 'NONE',  ( -11.05000000000000249, 2.500000000000000000, -6.148780366869522673 ) ) ;
#74622=VECTOR ( 'NONE', #68450, 1000.000000000000000 ) ;
#74624=ORIENTED_EDGE ( 'NONE', *, *, #114161, .F. ) ;
#74626=ORIENTED_EDGE ( 'NONE', *, *, #58941, .F. ) ;
#74627=ORIENTED_EDGE ( 'NONE', *, *, #75726, .T. ) ;
#74628=CARTESIAN_POINT ( 'NONE',  ( 0.6499999999999561684, 12.50000000000000000, -1.883746621131363375 ) ) ;
#74629=LINE ( 'NONE', #96190, #93807 ) ;
#74630=CIRCLE ( 'NONE', #18188, 0.1000000000000002554 ) ;
#74631=LINE ( 'NONE', #61609, #17171 ) ;
#74632=VECTOR ( 'NONE', #578, 1000.000000000000000 ) ;
#74633=DIRECTION ( 'NONE',  ( -0.000000000000000000, -1.000000000000000000, -0.000000000000000000 ) ) ;
#74634=CARTESIAN_POINT ( 'NONE',  ( 5.399999999999932854, 2.500000000000000000, 4.922947341949748257 ) ) ;
#74635=ORIENTED_EDGE ( 'NONE', *, *, #22269, .T. ) ;
#74636=CARTESIAN_POINT ( 'NONE',  ( 11.24999999999990941, 12.50000000000000000, 7.188010851410848723 ) ) ;
#74637=CARTESIAN_POINT ( 'NONE',  ( 13.94999999999989448, 12.50000000000000000, -2.511473670974877948 ) ) ;
#74638=CONICAL_SURFACE ( 'NONE', #45409, 0.1000000000000000472, 0.003490658503988666988 ) ;
#74640=DIRECTION ( 'NONE',  ( -0.000000000000000000, 1.000000000000000000, -0.000000000000000000 ) ) ;
#74641=VERTEX_POINT ( 'NONE', #127858 ) ;
#74642=ORIENTED_EDGE ( 'NONE', *, *, #105540, .F. ) ;
#74643=ORIENTED_EDGE ( 'NONE', *, *, #108026, .T. ) ;
#74644=DIRECTION ( 'NONE',  ( 0.000000000000000000, 0.000000000000000000, 1.000000000000000000 ) ) ;
#74645=AXIS2_PLACEMENT_3D ( 'NONE', #85097, #18771, #99281 ) ;
#74646=AXIS2_PLACEMENT_3D ( 'NONE', #54251, #114449, #25409 ) ;
#74647=FACE_OUTER_BOUND ( 'NONE', #69525, .T. ) ;
#74648=PLANE ( 'NONE',  #71171 ) ;
#74649=AXIS2_PLACEMENT_3D ( 'NONE', #107558, #49305, #46703 ) ;
#74650=EDGE_CURVE ( 'NONE', #3051, #95827, #16512, .T. ) ;
#74651=VERTEX_POINT ( 'NONE', #108851 ) ;
#74652=CARTESIAN_POINT ( 'NONE',  ( 10.79999999999991012, 2.500000000000000000, 4.330127018922196314 ) ) ;
#74653=CARTESIAN_POINT ( 'NONE',  ( -13.54999999999998828, 2.500000000000000000, 1.818653347947325472 ) ) ;
#74654=EDGE_CURVE ( 'NONE', #119878, #27277, #116370, .T. ) ;
#74655=DIRECTION ( 'NONE',  ( 0.000000000000000000, 0.000000000000000000, -1.000000000000000000 ) ) ;
#74656=CARTESIAN_POINT ( 'NONE',  ( 2.099999999999947686, 2.500000000000000000, 4.922947341949748257 ) ) ;
#74657=DIRECTION ( 'NONE',  ( -0.000000000000000000, -1.000000000000000000, -0.000000000000000000 ) ) ;
#74658=ADVANCED_FACE ( 'NONE', ( #129185 ), #122861, .T. ) ;
#74659=EDGE_LOOP ( 'NONE', ( #12027, #83366, #73986, #9336 ) ) ;
#74660=DIRECTION ( 'NONE',  ( -0.000000000000000000, 1.000000000000000000, -0.000000000000000000 ) ) ;
#74662=EDGE_CURVE ( 'NONE', #52767, #91667, #56231, .T. ) ;
#74663=ADVANCED_FACE ( 'NONE', ( #31602 ), #30933, .T. ) ;
#74664=ORIENTED_EDGE ( 'NONE', *, *, #125947, .F. ) ;
#74665=EDGE_CURVE ( 'NONE', #59178, #58192, #22446, .T. ) ;
#74666=DIRECTION ( 'NONE',  ( -0.000000000000000000, 1.000000000000000000, -0.000000000000000000 ) ) ;
#74667=EDGE_CURVE ( 'NONE', #28644, #59160, #116585, .T. ) ;
#74668=ADVANCED_FACE ( 'NONE', ( #72181 ), #127074, .T. ) ;
#74669=FACE_BOUND ( 'NONE', #28204, .T. ) ;
#74670=CIRCLE ( 'NONE', #124853, 0.06509327318403745899 ) ;
#74671=DIRECTION ( 'NONE',  ( -4.274815082592931898E-19, -0.9999939076577903929, -0.003490651415223739937 ) ) ;
#74672=CARTESIAN_POINT ( 'NONE',  ( -7.500000000000001776, -2.500000000000000000, 9.000000000000001776 ) ) ;
#74673=AXIS2_PLACEMENT_3D ( 'NONE', #99542, #28216, #128370 ) ;
#74674=CARTESIAN_POINT ( 'NONE',  ( 11.04999999999991012, 2.500000000000000000, -1.818653347947326138 ) ) ;
#74675=VERTEX_POINT ( 'NONE', #91164 ) ;
#74676=CIRCLE ( 'NONE', #91393, 0.1000000000000002554 ) ;
#74678=CARTESIAN_POINT ( 'NONE',  ( -4.150000000000025224, 12.50000000000000000, -1.472243186433550122 ) ) ;
#74679=DIRECTION ( 'NONE',  ( 0.000000000000000000, 1.000000000000000000, 0.000000000000000000 ) ) ;
#74680=EDGE_CURVE ( 'NONE', #73467, #97281, #41441, .T. ) ;
#74681=CIRCLE ( 'NONE', #18328, 0.06509327318403745899 ) ;
#74682=CARTESIAN_POINT ( 'NONE',  ( 15.83209681635555910, -2.500000000000000000, -5.404881881984148428 ) ) ;
#74683=AXIS2_PLACEMENT_3D ( 'NONE', #103863, #52818, #113024 ) ;
#74684=CARTESIAN_POINT ( 'NONE',  ( -10.84999999999999964, 12.50000000000000000, 1.407149913249508000 ) ) ;
#74685=VERTEX_POINT ( 'NONE', #101637 ) ;
#74686=DIRECTION ( 'NONE',  ( -4.274815082592931898E-19, -0.9999939076577903929, -0.003490651415223739937 ) ) ;
#74687=AXIS2_PLACEMENT_3D ( 'NONE', #103477, #62908, #73362 ) ;
#74688=FACE_OUTER_BOUND ( 'NONE', #27992, .T. ) ;
#74689=ORIENTED_EDGE ( 'NONE', *, *, #72, .T. ) ;
#74690=DIRECTION ( 'NONE',  ( -4.274815082592931898E-19, -0.9999939076577903929, -0.003490651415223739937 ) ) ;
#74691=AXIS2_PLACEMENT_3D ( 'NONE', #2447, #50286, #43070 ) ;
#74692=VERTEX_POINT ( 'NONE', #11950 ) ;
#74693=FACE_BOUND ( 'NONE', #76962, .T. ) ;
#74694=CARTESIAN_POINT ( 'NONE',  ( -12.49999999999995914, 2.500000000000000000, 1.843143693225357538E-15 ) ) ;
#74695=AXIS2_PLACEMENT_3D ( 'NONE', #31782, #71700, #61899 ) ;
#74696=CIRCLE ( 'NONE', #83033, 0.06509327318403745899 ) ;
#74697=VERTEX_POINT ( 'NONE', #81353 ) ;
#74698=CARTESIAN_POINT ( 'NONE',  ( 12.49999999999990230, 12.50000000000000000, -0.6277270498435166823 ) ) ;
#74700=ORIENTED_EDGE ( 'NONE', *, *, #63426, .T. ) ;
#74701=VERTEX_POINT ( 'NONE', #40129 ) ;
#74704=CARTESIAN_POINT ( 'NONE',  ( -12.89999999999999147, 2.500000000000000000, 1.843143693225357538E-15 ) ) ;
#74705=DIRECTION ( 'NONE',  ( 0.000000000000000000, 0.000000000000000000, 1.000000000000000000 ) ) ;
#74706=DIRECTION ( 'NONE',  ( 0.000000000000000000, 0.000000000000000000, -1.000000000000000000 ) ) ;
#74708=ADVANCED_FACE ( 'NONE', ( #91807 ), #14172, .T. ) ;
#74709=DIRECTION ( 'NONE',  ( 0.000000000000000000, 0.000000000000000000, 1.000000000000000000 ) ) ;
#74710=CIRCLE ( 'NONE', #14051, 0.06509327318403745899 ) ;
#74711=EDGE_CURVE ( 'NONE', #99143, #30225, #64359, .T. ) ;
#74712=VERTEX_POINT ( 'NONE', #111429 ) ;
#74713=ADVANCED_FACE ( 'NONE', ( #10634 ), #81106, .T. ) ;
#74714=ORIENTED_EDGE ( 'NONE', *, *, #5126, .F. ) ;
#74715=CARTESIAN_POINT ( 'NONE',  ( -8.150000000000012790, 2.500000000000000000, -2.511473670974877948 ) ) ;
#74716=DIRECTION ( 'NONE',  ( -0.000000000000000000, -1.000000000000000000, -0.000000000000000000 ) ) ;
#74717=DIRECTION ( 'NONE',  ( 0.000000000000000000, 0.000000000000000000, -1.000000000000000000 ) ) ;
#74718=FACE_OUTER_BOUND ( 'NONE', #92984, .T. ) ;
#74719=EDGE_LOOP ( 'NONE', ( #13875, #84989, #18263, #117509 ) ) ;
#74720=ORIENTED_EDGE ( 'NONE', *, *, #18722, .F. ) ;
#74721=CARTESIAN_POINT ( 'NONE',  ( 3.349999999999945466, 12.50000000000000000, -2.165063509461101710 ) ) ;
#74722=EDGE_LOOP ( 'NONE', ( #120486, #4322, #5059, #822 ) ) ;
#74723=ADVANCED_FACE ( 'NONE', ( #12587 ), #52519, .T. ) ;
#74724=DIRECTION ( 'NONE',  ( -0.000000000000000000, -1.000000000000000000, -0.000000000000000000 ) ) ;
#74725=CARTESIAN_POINT ( 'NONE',  ( -10.40000000000000213, 2.500000000000000000, -0.5928203230275541635 ) ) ;
#74726=EDGE_CURVE ( 'NONE', #106877, #117445, #5759, .T. ) ;
#74727=VERTEX_POINT ( 'NONE', #80711 ) ;
#74728=CARTESIAN_POINT ( 'NONE',  ( 9.349999999999919709, 2.500000000000000000, -6.048780366869526581 ) ) ;
#74729=CARTESIAN_POINT ( 'NONE',  ( -9.150000000000005684, 12.50000000000000000, 6.495190528383297135 ) ) ;
#74730=CIRCLE ( 'NONE', #95658, 0.09999999999999982514 ) ;
#74731=EDGE_CURVE ( 'NONE', #41978, #90278, #119980, .T. ) ;
#74732=DIRECTION ( 'NONE',  ( -0.000000000000000000, 1.000000000000000000, -0.000000000000000000 ) ) ;
#74733=VECTOR ( 'NONE', #64979, 1000.000000000000000 ) ;
#74734=EDGE_CURVE ( 'NONE', #121834, #104854, #30977, .T. ) ;
#74735=DIRECTION ( 'NONE',  ( 0.000000000000000000, 0.000000000000000000, -1.000000000000000000 ) ) ;
#74736=LINE ( 'NONE', #7260, #101780 ) ;
#74737=DIRECTION ( 'NONE',  ( 0.000000000000000000, 1.000000000000000000, 0.000000000000000000 ) ) ;
#74739=CARTESIAN_POINT ( 'NONE',  ( 4.599999999999938360, 12.50000000000000000, -2.276824562219559311E-15 ) ) ;
#74740=DIRECTION ( 'NONE',  ( 0.000000000000000000, 0.000000000000000000, -1.000000000000000000 ) ) ;
#74741=EDGE_CURVE ( 'NONE', #109874, #77490, #22531, .T. ) ;
#74742=AXIS2_PLACEMENT_3D ( 'NONE', #15570, #106535, #55518 ) ;
#74743=CIRCLE ( 'NONE', #124916, 0.09999999999999982514 ) ;
#74744=ORIENTED_EDGE ( 'NONE', *, *, #92553, .T. ) ;
#74745=EDGE_LOOP ( 'NONE', ( #66617, #80258, #21013, #28328 ) ) ;
#74746=AXIS2_PLACEMENT_3D ( 'NONE', #64921, #114040, #115967 ) ;
#74747=ORIENTED_EDGE ( 'NONE', *, *, #109467, .F. ) ;
#74748=DIRECTION ( 'NONE',  ( 0.000000000000000000, 0.000000000000000000, -1.000000000000000000 ) ) ;
#74749=ORIENTED_EDGE ( 'NONE', *, *, #98076, .T. ) ;
#74750=CARTESIAN_POINT ( 'NONE',  ( 0.8499999999999550138, 2.500000000000000000, -5.702370205355749455 ) ) ;
#74751=ORIENTED_EDGE ( 'NONE', *, *, #110678, .T. ) ;
#74752=ORIENTED_EDGE ( 'NONE', *, *, #92889, .T. ) ;
#74753=EDGE_LOOP ( 'NONE', ( #25023, #10895, #5044, #26779 ) ) ;
#74754=DIRECTION ( 'NONE',  ( 0.000000000000000000, 0.000000000000000000, 1.000000000000000000 ) ) ;
#74755=AXIS2_PLACEMENT_3D ( 'NONE', #74966, #114878, #76264 ) ;
#74756=AXIS2_PLACEMENT_3D ( 'NONE', #30945, #41410, #11921 ) ;
#74758=DIRECTION ( 'NONE',  ( 0.000000000000000000, 1.000000000000000000, 0.000000000000000000 ) ) ;
#74759=DIRECTION ( 'NONE',  ( 0.000000000000000000, -0.9999939076577903929, 0.003490651415223739937 ) ) ;
#74760=DIRECTION ( 'NONE',  ( 0.000000000000000000, 1.000000000000000000, 0.000000000000000000 ) ) ;
#74761=ADVANCED_FACE ( 'NONE', ( #70015 ), #38637, .T. ) ;
#74762=ORIENTED_EDGE ( 'NONE', *, *, #52108, .F. ) ;
#74763=DIRECTION ( 'NONE',  ( 0.000000000000000000, 0.000000000000000000, -1.000000000000000000 ) ) ;
#74764=EDGE_LOOP ( 'NONE', ( #39979, #91496 ) ) ;
#74765=CIRCLE ( 'NONE', #129071, 0.09999999999999982514 ) ;
#74766=EDGE_LOOP ( 'NONE', ( #32650, #26670, #42555, #23876 ) ) ;
#74767=EDGE_LOOP ( 'NONE', ( #126227, #47288 ) ) ;
#74768=CONICAL_SURFACE ( 'NONE', #74855, 0.1000000000000000472, 0.003490658503988666988 ) ;
#74769=CARTESIAN_POINT ( 'NONE',  ( -1.050000000000037792, 12.50000000000000000, 1.883746621131358934 ) ) ;
#74770=ORIENTED_EDGE ( 'NONE', *, *, #56900, .T. ) ;
#74771=ORIENTED_EDGE ( 'NONE', *, *, #74264, .T. ) ;
#74772=VERTEX_POINT ( 'NONE', #109279 ) ;
#74773=CONICAL_SURFACE ( 'NONE', #3656, 0.1000000000000002554, 0.003490658503988666988 ) ;
#74774=CIRCLE ( 'NONE', #62262, 0.09999999999999999167 ) ;
#74775=CARTESIAN_POINT ( 'NONE',  ( -3.642919299551294898E-14, 12.50000000000000000, 0.6928203230275518099 ) ) ;
#74776=DIRECTION ( 'NONE',  ( 0.000000000000000000, -0.9999939076577903929, 0.003490651415223739937 ) ) ;
#74777=CARTESIAN_POINT ( 'NONE',  ( -1.250000000000035749, 12.50000000000000000, -7.188010851410854052 ) ) ;
#74778=AXIS2_PLACEMENT_3D ( 'NONE', #65131, #86060, #124718 ) ;
#74779=EDGE_CURVE ( 'NONE', #41136, #17717, #95673, .T. ) ;
#74780=CARTESIAN_POINT ( 'NONE',  ( 1.899999999999951283, 2.500000000000000000, 0.4464101615137736623 ) ) ;
#74781=DIRECTION ( 'NONE',  ( 0.000000000000000000, 0.000000000000000000, -1.000000000000000000 ) ) ;
#74782=CARTESIAN_POINT ( 'NONE',  ( 8.949999999999917577, 12.50000000000000000, -2.446380397790840266 ) ) ;
#74783=ORIENTED_EDGE ( 'NONE', *, *, #14551, .F. ) ;
#74784=AXIS2_PLACEMENT_3D ( 'NONE', #25132, #96440, #6129 ) ;
#74785=CARTESIAN_POINT ( 'NONE',  ( 9.599999999999914380, 2.500000000000000000, 5.122947341949749323 ) ) ;
#74786=VECTOR ( 'NONE', #80851, 1000.000000000000000 ) ;
#74787=ORIENTED_EDGE ( 'NONE', *, *, #112257, .T. ) ;
#74788=AXIS2_PLACEMENT_3D ( 'NONE', #59567, #39281, #70638 ) ;
#74789=PLANE ( 'NONE',  #40140 ) ;
#74790=ORIENTED_EDGE ( 'NONE', *, *, #77206, .F. ) ;
#74791=CARTESIAN_POINT ( 'NONE',  ( -11.69999999999999574, 2.500000000000000000, 4.330127018922196314 ) ) ;
#74792=ORIENTED_EDGE ( 'NONE', *, *, #20197, .F. ) ;
#74793=CIRCLE ( 'NONE', #18341, 0.1000000000000002554 ) ;
#74794=EDGE_CURVE ( 'NONE', #83303, #52300, #58903, .T. ) ;
#74795=EDGE_LOOP ( 'NONE', ( #97941, #44337 ) ) ;
#74796=FACE_OUTER_BOUND ( 'NONE', #21041, .T. ) ;
#74797=CARTESIAN_POINT ( 'NONE',  ( 4.349999999999941025, 2.500000000000000000, -6.248780366869526759 ) ) ;
#74798=AXIS2_PLACEMENT_3D ( 'NONE', #60467, #878, #90535 ) ;
#74799=AXIS2_PLACEMENT_3D ( 'NONE', #17154, #106224, #105581 ) ;
#74800=FACE_OUTER_BOUND ( 'NONE', #102366, .T. ) ;
#74801=DIRECTION ( 'NONE',  ( 0.000000000000000000, 0.000000000000000000, 1.000000000000000000 ) ) ;
#74802=ORIENTED_EDGE ( 'NONE', *, *, #2983, .T. ) ;
#74803=DIRECTION ( 'NONE',  ( -0.000000000000000000, -1.000000000000000000, -0.000000000000000000 ) ) ;
#74804=DIRECTION ( 'NONE',  ( 0.000000000000000000, 0.000000000000000000, 1.000000000000000000 ) ) ;
#74805=CARTESIAN_POINT ( 'NONE',  ( -11.04999999999999893, 2.500000000000000000, 1.818653347947321475 ) ) ;
#74806=DIRECTION ( 'NONE',  ( 0.000000000000000000, 1.000000000000000000, 0.000000000000000000 ) ) ;
#74807=CARTESIAN_POINT ( 'NONE',  ( 1.849999999999950129, 12.50000000000000000, -6.841600689897078702 ) ) ;
#74808=VERTEX_POINT ( 'NONE', #57616 ) ;
#74809=EDGE_LOOP ( 'NONE', ( #21662, #53944 ) ) ;
#74811=DIRECTION ( 'NONE',  ( 0.000000000000000000, 1.000000000000000000, 0.000000000000000000 ) ) ;
#74812=DIRECTION ( 'NONE',  ( -0.000000000000000000, 1.000000000000000000, -0.000000000000000000 ) ) ;
#74813=EDGE_CURVE ( 'NONE', #87854, #91937, #55953, .T. ) ;
#74814=VECTOR ( 'NONE', #63291, 1000.000000000000000 ) ;
#74816=LINE ( 'NONE', #24424, #82434 ) ;
#74817=CARTESIAN_POINT ( 'NONE',  ( 2.499999999999983569, 2.500000000000000000, -2.276824562219559311E-15 ) ) ;
#74818=LINE ( 'NONE', #14587, #89985 ) ;
#74819=DIRECTION ( 'NONE',  ( 0.000000000000000000, 0.000000000000000000, 1.000000000000000000 ) ) ;
#74820=ORIENTED_EDGE ( 'NONE', *, *, #47603, .T. ) ;
#74821=CIRCLE ( 'NONE', #7907, 0.06509327318403745899 ) ;
#74822=AXIS2_PLACEMENT_3D ( 'NONE', #63563, #102813, #30895 ) ;
#74823=CARTESIAN_POINT ( 'NONE',  ( -2.300000000000033573, 2.500000000000000000, -3.983716857408426293 ) ) ;
#74824=DIRECTION ( 'NONE',  ( -4.274815082592931898E-19, -0.9999939076577903929, -0.003490651415223739937 ) ) ;
#74825=ORIENTED_EDGE ( 'NONE', *, *, #96889, .F. ) ;
#74826=EDGE_CURVE ( 'NONE', #87658, #69489, #129146, .T. ) ;
#74827=ADVANCED_FACE ( 'NONE', ( #19618 ), #49096, .T. ) ;
#74828=ADVANCED_FACE ( 'NONE', ( #7847 ), #8486, .T. ) ;
#74829=EDGE_CURVE ( 'NONE', #90721, #48277, #10084, .T. ) ;
#74830=AXIS2_PLACEMENT_3D ( 'NONE', #17262, #57217, #127263 ) ;
#74831=DIRECTION ( 'NONE',  ( -0.000000000000000000, 1.000000000000000000, -0.000000000000000000 ) ) ;
#74832=CIRCLE ( 'NONE', #127073, 0.1000000000000002554 ) ;
#74833=AXIS2_PLACEMENT_3D ( 'NONE', #107989, #10436, #28150 ) ;
#74834=EDGE_LOOP ( 'NONE', ( #106210, #57753, #2075, #23205 ) ) ;
#74835=EDGE_CURVE ( 'NONE', #37927, #59380, #58121, .T. ) ;
#74836=DIRECTION ( 'NONE',  ( 0.000000000000000000, -0.9999939076577903929, 0.003490651415223739937 ) ) ;
#74837=ORIENTED_EDGE ( 'NONE', *, *, #8656, .T. ) ;
#74838=DIRECTION ( 'NONE',  ( -0.000000000000000000, 1.000000000000000000, -0.000000000000000000 ) ) ;
#74839=CARTESIAN_POINT ( 'NONE',  ( 10.64999999999991331, 2.500000000000000000, -1.718653347947325827 ) ) ;
#74840=ADVANCED_FACE ( 'NONE', ( #79198 ), #26808, .T. ) ;
#74841=DIRECTION ( 'NONE',  ( 0.000000000000000000, 0.000000000000000000, -1.000000000000000000 ) ) ;
#74842=ORIENTED_EDGE ( 'NONE', *, *, #81555, .F. ) ;
#74843=ADVANCED_FACE ( 'NONE', ( #29443 ), #93701, .T. ) ;
#74844=CONICAL_SURFACE ( 'NONE', #58125, 0.1000000000000000472, 0.003490658503988666988 ) ;
#74845=FACE_OUTER_BOUND ( 'NONE', #52352, .T. ) ;
#74846=EDGE_CURVE ( 'NONE', #49848, #75839, #5857, .T. ) ;
#74848=CIRCLE ( 'NONE', #45615, 0.09999999999999982514 ) ;
#74849=ADVANCED_FACE ( 'NONE', ( #117142 ), #100117, .T. ) ;
#74850=ORIENTED_EDGE ( 'NONE', *, *, #34460, .T. ) ;
#74851=CARTESIAN_POINT ( 'NONE',  ( -5.450000000000019718, 12.50000000000000000, 6.430097255199259010 ) ) ;
#74852=VECTOR ( 'NONE', #6388, 1000.000000000000000 ) ;
#74853=VERTEX_POINT ( 'NONE', #68064 ) ;
#74854=ORIENTED_EDGE ( 'NONE', *, *, #41147, .F. ) ;
#74855=AXIS2_PLACEMENT_3D ( 'NONE', #79433, #99065, #129195 ) ;
#74856=CARTESIAN_POINT ( 'NONE',  ( -5.850000000000022737, 2.500000000000000000, -2.065063509461102065 ) ) ;
#74857=DIRECTION ( 'NONE',  ( 0.000000000000000000, -0.9999939076577903929, 0.003490651415223739937 ) ) ;
#74858=ORIENTED_EDGE ( 'NONE', *, *, #11743, .T. ) ;
#74859=VECTOR ( 'NONE', #74759, 1000.000000000000000 ) ;
#74860=DIRECTION ( 'NONE',  ( -0.000000000000000000, 1.000000000000000000, -0.000000000000000000 ) ) ;
#74861=DIRECTION ( 'NONE',  ( -4.274815082592931898E-19, -0.9999939076577903929, -0.003490651415223739937 ) ) ;
#74862=AXIS2_PLACEMENT_3D ( 'NONE', #77966, #30830, #108070 ) ;
#74863=ORIENTED_EDGE ( 'NONE', *, *, #84487, .F. ) ;
#74864=DIRECTION ( 'NONE',  ( 0.000000000000000000, 0.000000000000000000, 1.000000000000000000 ) ) ;
#74865=LINE ( 'NONE', #115393, #76495 ) ;
#74866=CIRCLE ( 'NONE', #18428, 0.06509327318403745899 ) ;
#74867=CARTESIAN_POINT ( 'NONE',  ( 0.6499999999999543920, 2.500000000000000000, 6.148780366869520897 ) ) ;
#74868=CARTESIAN_POINT ( 'NONE',  ( -13.29999999999999005, 2.500000000000000000, 1.843143693225357538E-15 ) ) ;
#74869=DIRECTION ( 'NONE',  ( -0.000000000000000000, -1.000000000000000000, -0.000000000000000000 ) ) ;
#74870=LINE ( 'NONE', #25760, #45176 ) ;
#74871=AXIS2_PLACEMENT_3D ( 'NONE', #16424, #87121, #125740 ) ;
#74872=DIRECTION ( 'NONE',  ( -0.000000000000000000, -1.000000000000000000, -0.000000000000000000 ) ) ;
#74873=VERTEX_POINT ( 'NONE', #37338 ) ;
#74874=EDGE_LOOP ( 'NONE', ( #16901, #4334 ) ) ;
#74875=ORIENTED_EDGE ( 'NONE', *, *, #90177, .F. ) ;
#74876=VERTEX_POINT ( 'NONE', #128294 ) ;
#74877=CARTESIAN_POINT ( 'NONE',  ( -2.900000000000030109, 2.500000000000000000, 0.7928203230275495672 ) ) ;
#74879=DIRECTION ( 'NONE',  ( 0.000000000000000000, 0.000000000000000000, -1.000000000000000000 ) ) ;
#74880=AXIS2_PLACEMENT_3D ( 'NONE', #122517, #93066, #91120 ) ;
#74881=VERTEX_POINT ( 'NONE', #118451 ) ;
#74882=FACE_BOUND ( 'NONE', #23941, .T. ) ;
#74883=DIRECTION ( 'NONE',  ( 0.000000000000000000, -0.000000000000000000, 1.000000000000000000 ) ) ;
#74884=CARTESIAN_POINT ( 'NONE',  ( -1.250000000000036193, 12.50000000000000000, 1.472243186433545459 ) ) ;
#74885=EDGE_CURVE ( 'NONE', #73184, #63382, #108280, .T. ) ;
#74886=CARTESIAN_POINT ( 'NONE',  ( 8.299999999999922551, 12.50000000000000000, -0.06509327318403980434 ) ) ;
#74887=AXIS2_PLACEMENT_3D ( 'NONE', #30685, #66870, #127105 ) ;
#74888=CONICAL_SURFACE ( 'NONE', #112550, 0.09999999999999982514, 0.003490658503988666988 ) ;
#74889=CARTESIAN_POINT ( 'NONE',  ( -3.950000000000025491, 2.500000000000000000, 6.048780366869521252 ) ) ;
#74890=EDGE_CURVE ( 'NONE', #27457, #111073, #129243, .T. ) ;
#74891=FACE_OUTER_BOUND ( 'NONE', #102328, .T. ) ;
#74892=DIRECTION ( 'NONE',  ( 0.000000000000000000, 1.000000000000000000, 0.000000000000000000 ) ) ;
#74893=CARTESIAN_POINT ( 'NONE',  ( 12.09999999999990550, 12.50000000000000000, -5.022947341949754119 ) ) ;
#74894=DIRECTION ( 'NONE',  ( -0.000000000000000000, -1.000000000000000000, -0.000000000000000000 ) ) ;
#74895=DIRECTION ( 'NONE',  ( 0.000000000000000000, 1.000000000000000000, 0.000000000000000000 ) ) ;
#74896=DIRECTION ( 'NONE',  ( 0.000000000000000000, 0.000000000000000000, 1.000000000000000000 ) ) ;
#74897=EDGE_CURVE ( 'NONE', #40079, #118967, #99972, .T. ) ;
#74898=ORIENTED_EDGE ( 'NONE', *, *, #108976, .F. ) ;
#74899=VERTEX_POINT ( 'NONE', #112517 ) ;
#74900=ORIENTED_EDGE ( 'NONE', *, *, #46316, .T. ) ;
#74901=VERTEX_POINT ( 'NONE', #21552 ) ;
#74902=DIRECTION ( 'NONE',  ( -0.000000000000000000, 1.000000000000000000, -0.000000000000000000 ) ) ;
#74903=ORIENTED_EDGE ( 'NONE', *, *, #88238, .F. ) ;
#74904=CONICAL_SURFACE ( 'NONE', #56103, 0.1000000000000000472, 0.003490658503988666988 ) ;
#74905=DIRECTION ( 'NONE',  ( 0.000000000000000000, -0.000000000000000000, 1.000000000000000000 ) ) ;
#74906=ORIENTED_EDGE ( 'NONE', *, *, #53539, .T. ) ;
#74907=ORIENTED_EDGE ( 'NONE', *, *, #29790, .T. ) ;
#74908=AXIS2_PLACEMENT_3D ( 'NONE', #81251, #113931, #112001 ) ;
#74909=CARTESIAN_POINT ( 'NONE',  ( 10.79999999999991012, 12.50000000000000000, -4.395220292106239768 ) ) ;
#74910=CIRCLE ( 'NONE', #26787, 0.06509327318403743123 ) ;
#74911=VECTOR ( 'NONE', #120323, 1000.000000000000000 ) ;
#74912=CARTESIAN_POINT ( 'NONE',  ( 8.949999999999919353, 12.50000000000000000, -6.083687093685488989 ) ) ;
#74913=DIRECTION ( 'NONE',  ( -4.274815082592931898E-19, -0.9999939076577903929, -0.003490651415223739937 ) ) ;
#74914=PLANE ( 'NONE',  #64297 ) ;
#74915=ORIENTED_EDGE ( 'NONE', *, *, #5457, .F. ) ;
#74916=AXIS2_PLACEMENT_3D ( 'NONE', #25486, #83776, #94237 ) ;
#74917=VERTEX_POINT ( 'NONE', #32691 ) ;
#74918=CIRCLE ( 'NONE', #112661, 0.1000000000000002554 ) ;
#74919=ORIENTED_EDGE ( 'NONE', *, *, #56962, .F. ) ;
#74920=LINE ( 'NONE', #17754, #44769 ) ;
#74921=ORIENTED_EDGE ( 'NONE', *, *, #90400, .F. ) ;
#74922=PLANE ( 'NONE',  #123621 ) ;
#74923=EDGE_LOOP ( 'NONE', ( #109521, #3028 ) ) ;
#74924=VERTEX_POINT ( 'NONE', #52953 ) ;
#74925=CIRCLE ( 'NONE', #18478, 0.09999999999999982514 ) ;
#74926=DIRECTION ( 'NONE',  ( -0.000000000000000000, 1.000000000000000000, -0.000000000000000000 ) ) ;
#74927=AXIS2_PLACEMENT_3D ( 'NONE', #104095, #7165, #47121 ) ;
#74928=DIRECTION ( 'NONE',  ( -0.000000000000000000, -1.000000000000000000, -0.000000000000000000 ) ) ;
#74929=CARTESIAN_POINT ( 'NONE',  ( 7.899999999999924860, 12.50000000000000000, 4.330127018922196314 ) ) ;
#74931=DIRECTION ( 'NONE',  ( 0.000000000000000000, 0.000000000000000000, 1.000000000000000000 ) ) ;
#74932=VERTEX_POINT ( 'NONE', #92882 ) ;
#74933=DIRECTION ( 'NONE',  ( 0.000000000000000000, 0.000000000000000000, 1.000000000000000000 ) ) ;
#74934=CONICAL_SURFACE ( 'NONE', #106235, 0.1000000000000002554, 0.003490658503988666988 ) ;
#74935=EDGE_LOOP ( 'NONE', ( #124122, #41801, #5767, #18643 ) ) ;
#74936=FACE_OUTER_BOUND ( 'NONE', #28517, .T. ) ;
#74937=EDGE_LOOP ( 'NONE', ( #84384, #114027, #84061, #2167 ) ) ;
#74938=DIRECTION ( 'NONE',  ( 0.000000000000000000, 0.000000000000000000, 1.000000000000000000 ) ) ;
#74939=CARTESIAN_POINT ( 'NONE',  ( -4.999999999999986677, 12.50000000000000000, 4.265033745738159077 ) ) ;
#74940=EDGE_CURVE ( 'NONE', #20160, #13428, #3817, .T. ) ;
#74941=AXIS2_PLACEMENT_3D ( 'NONE', #101034, #52573, #42118 ) ;
#74942=DIRECTION ( 'NONE',  ( 0.000000000000000000, 1.000000000000000000, 0.000000000000000000 ) ) ;
#74943=ADVANCED_FACE ( 'NONE', ( #70647 ), #22623, .T. ) ;
#74944=DIRECTION ( 'NONE',  ( 0.000000000000000000, -0.000000000000000000, 1.000000000000000000 ) ) ;
#74945=EDGE_LOOP ( 'NONE', ( #29309, #84367, #106340, #23302 ) ) ;
#74946=CARTESIAN_POINT ( 'NONE',  ( 1.649999999999951505, 12.50000000000000000, -1.407149913249512663 ) ) ;
#74947=VECTOR ( 'NONE', #1849, 1000.000000000000000 ) ;
#74949=DIRECTION ( 'NONE',  ( 0.000000000000000000, 0.000000000000000000, 1.000000000000000000 ) ) ;
#74950=ORIENTED_EDGE ( 'NONE', *, *, #128959, .T. ) ;
#74951=ORIENTED_EDGE ( 'NONE', *, *, #62139, .T. ) ;
#74952=EDGE_CURVE ( 'NONE', #125908, #79919, #113148, .T. ) ;
#74953=VERTEX_POINT ( 'NONE', #30751 ) ;
#74954=CARTESIAN_POINT ( 'NONE',  ( -4.550000000000022915, 12.50000000000000000, 6.560283801567334372 ) ) ;
#74955=DIRECTION ( 'NONE',  ( 0.000000000000000000, 0.000000000000000000, -1.000000000000000000 ) ) ;
#74958=AXIS2_PLACEMENT_3D ( 'NONE', #74929, #43550, #25169 ) ;
#74959=DIRECTION ( 'NONE',  ( 0.000000000000000000, 0.000000000000000000, 1.000000000000000000 ) ) ;
#74960=DIRECTION ( 'NONE',  ( -0.000000000000000000, -1.000000000000000000, -0.000000000000000000 ) ) ;
#74961=CIRCLE ( 'NONE', #26842, 0.1000000000000002554 ) ;
#74962=VERTEX_POINT ( 'NONE', #110572 ) ;
#74963=DIRECTION ( 'NONE',  ( 0.000000000000000000, 1.000000000000000000, 0.000000000000000000 ) ) ;
#74964=EDGE_CURVE ( 'NONE', #99874, #36233, #43548, .T. ) ;
#74965=ORIENTED_EDGE ( 'NONE', *, *, #92853, .F. ) ;
#74966=CARTESIAN_POINT ( 'NONE',  ( -13.74999999999998934, 2.500000000000000000, 2.857883832488652853 ) ) ;
#74967=CARTESIAN_POINT ( 'NONE',  ( -12.09999999999999609, 12.50000000000000000, 4.330127018922196314 ) ) ;
#74968=DIRECTION ( 'NONE',  ( 0.000000000000000000, 0.000000000000000000, 1.000000000000000000 ) ) ;
#74969=EDGE_LOOP ( 'NONE', ( #22747, #103487 ) ) ;
#74970=ADVANCED_FACE ( 'NONE', ( #73232 ), #85288, .T. ) ;
#74971=AXIS2_PLACEMENT_3D ( 'NONE', #4179, #44124, #24487 ) ;
#74972=CIRCLE ( 'NONE', #12262, 0.1000000000000000472 ) ;
#74974=CARTESIAN_POINT ( 'NONE',  ( -6.450000000000016165, 2.500000000000000000, 6.841600689897072485 ) ) ;
#74975=ADVANCED_FACE ( 'NONE', ( #42497 ), #83062, .T. ) ;
#74976=EDGE_CURVE ( 'NONE', #122967, #25509, #56035, .T. ) ;
#74977=EDGE_CURVE ( 'NONE', #121192, #25178, #45597, .T. ) ;
#74978=EDGE_CURVE ( 'NONE', #77678, #58293, #92210, .T. ) ;
#74979=ORIENTED_EDGE ( 'NONE', *, *, #42173, .T. ) ;
#74980=FACE_OUTER_BOUND ( 'NONE', #125537, .T. ) ;
#74981=ORIENTED_EDGE ( 'NONE', *, *, #5274, .F. ) ;
#74982=EDGE_LOOP ( 'NONE', ( #24514, #38344 ) ) ;
#74983=DIRECTION ( 'NONE',  ( -0.000000000000000000, 1.000000000000000000, -0.000000000000000000 ) ) ;
#74984=EDGE_CURVE ( 'NONE', #90660, #12748, #70716, .T. ) ;
#74985=CIRCLE ( 'NONE', #54156, 0.06509327318403745899 ) ;
#74986=EDGE_CURVE ( 'NONE', #35098, #78690, #62133, .T. ) ;
#74987=ORIENTED_EDGE ( 'NONE', *, *, #96981, .T. ) ;
#74988=FACE_OUTER_BOUND ( 'NONE', #47506, .T. ) ;
#74989=LINE ( 'NONE', #114898, #121615 ) ;
#74990=PLANE ( 'NONE',  #100294 ) ;
#74991=ORIENTED_EDGE ( 'NONE', *, *, #9217, .T. ) ;
#74992=EDGE_CURVE ( 'NONE', #125017, #15707, #49809, .T. ) ;
#74993=AXIS2_PLACEMENT_3D ( 'NONE', #103312, #23451, #111167 ) ;
#74994=FACE_BOUND ( 'NONE', #86504, .T. ) ;
#74995=EDGE_CURVE ( 'NONE', #65424, #126915, #41399, .T. ) ;
#74996=VECTOR ( 'NONE', #99103, 1000.000000000000000 ) ;
#74997=CIRCLE ( 'NONE', #18561, 0.06509327318403745899 ) ;
#74998=DIRECTION ( 'NONE',  ( 0.000000000000000000, 0.000000000000000000, 1.000000000000000000 ) ) ;
#74999=CARTESIAN_POINT ( 'NONE',  ( 3.149999999999944400, 2.500000000000000000, 1.918653347947321564 ) ) ;
#75000=VERTEX_POINT ( 'NONE', #51027 ) ;
#75001=CARTESIAN_POINT ( 'NONE',  ( 3.949999999999942446, 2.500000000000000000, -2.411473670974877859 ) ) ;
#75002=DIRECTION ( 'NONE',  ( 0.000000000000000000, 0.000000000000000000, 1.000000000000000000 ) ) ;
#75003=EDGE_CURVE ( 'NONE', #33429, #18914, #63412, .T. ) ;
#75004=CIRCLE ( 'NONE', #43624, 0.06509327318403745899 ) ;
#75005=ORIENTED_EDGE ( 'NONE', *, *, #11658, .F. ) ;
#75006=AXIS2_PLACEMENT_3D ( 'NONE', #17603, #57547, #28084 ) ;
#75007=CIRCLE ( 'NONE', #39533, 0.06509327318403745899 ) ;
#75008=ORIENTED_EDGE ( 'NONE', *, *, #99561, .F. ) ;
#75009=ORIENTED_EDGE ( 'NONE', *, *, #117795, .T. ) ;
#75010=CARTESIAN_POINT ( 'NONE',  ( 5.849999999999932143, 2.500000000000000000, 1.572243186433545548 ) ) ;
#75011=DIRECTION ( 'NONE',  ( 0.000000000000000000, 1.000000000000000000, 0.000000000000000000 ) ) ;
#75012=CARTESIAN_POINT ( 'NONE',  ( -12.09999999999999432, 2.500000000000000000, 5.122947341949749323 ) ) ;
#75013=FACE_BOUND ( 'NONE', #67220, .T. ) ;
#75014=ORIENTED_EDGE ( 'NONE', *, *, #48546, .T. ) ;
#75016=CARTESIAN_POINT ( 'NONE',  ( 14.34999999999989662, 12.50000000000000000, 1.818653347947321475 ) ) ;
#75017=DIRECTION ( 'NONE',  ( -0.000000000000000000, 1.000000000000000000, -0.000000000000000000 ) ) ;
#75018=VECTOR ( 'NONE', #104579, 1000.000000000000000 ) ;
#75019=DIRECTION ( 'NONE',  ( 0.000000000000000000, -0.000000000000000000, 1.000000000000000000 ) ) ;
#75020=CARTESIAN_POINT ( 'NONE',  ( 3.099999999999945466, 12.50000000000000000, 0.4115034346978109769 ) ) ;
#75021=DIRECTION ( 'NONE',  ( 0.000000000000000000, -0.000000000000000000, 1.000000000000000000 ) ) ;
#75022=DIRECTION ( 'NONE',  ( 0.000000000000000000, 0.000000000000000000, -1.000000000000000000 ) ) ;
#75023=DIRECTION ( 'NONE',  ( 0.000000000000000000, 0.000000000000000000, -1.000000000000000000 ) ) ;
#75024=CIRCLE ( 'NONE', #58311, 0.09999999999999999167 ) ;
#75025=DIRECTION ( 'NONE',  ( 0.000000000000000000, 1.000000000000000000, 0.000000000000000000 ) ) ;
#75026=ORIENTED_EDGE ( 'NONE', *, *, #57908, .T. ) ;
#75027=ORIENTED_EDGE ( 'NONE', *, *, #52894, .T. ) ;
#75028=VERTEX_POINT ( 'NONE', #111871 ) ;
#75029=VERTEX_POINT ( 'NONE', #40570 ) ;
#75030=EDGE_LOOP ( 'NONE', ( #95181, #15709, #108741, #125981 ) ) ;
#75031=CARTESIAN_POINT ( 'NONE',  ( 10.39999999999991154, 12.50000000000000000, -3.637306695894650055 ) ) ;
#75032=CARTESIAN_POINT ( 'NONE',  ( -2.500000000000032863, 2.500000000000000000, 4.922947341949748257 ) ) ;
#75034=FACE_BOUND ( 'NONE', #101969, .T. ) ;
#75035=FACE_OUTER_BOUND ( 'NONE', #108890, .T. ) ;
#75036=EDGE_CURVE ( 'NONE', #37274, #942, #100737, .T. ) ;
#75037=CIRCLE ( 'NONE', #47862, 0.09999999999999982514 ) ;
#75038=DIRECTION ( 'NONE',  ( 0.000000000000000000, 0.000000000000000000, 1.000000000000000000 ) ) ;
#75039=ADVANCED_FACE ( 'NONE', ( #22218 ), #112493, .T. ) ;
#75040=EDGE_LOOP ( 'NONE', ( #37201, #112476 ) ) ;
#75041=CARTESIAN_POINT ( 'NONE',  ( 4.999999999999936939, 12.50000000000000000, -3.572213422710612374 ) ) ;
#75042=CARTESIAN_POINT ( 'NONE',  ( 9.599999999999914380, 2.500000000000000000, -4.230127018922201998 ) ) ;
#75043=DIRECTION ( 'NONE',  ( -4.274815082592931898E-19, -0.9999939076577903929, -0.003490651415223739937 ) ) ;
#75044=EDGE_LOOP ( 'NONE', ( #83290, #26214 ) ) ;
#75045=CONICAL_SURFACE ( 'NONE', #18608, 0.1000000000000002554, 0.003490658503988666988 ) ;
#75046=DIRECTION ( 'NONE',  ( 0.000000000000000000, -0.9999939076577903929, 0.003490651415223739937 ) ) ;
#75047=AXIS2_PLACEMENT_3D ( 'NONE', #37335, #117784, #117139 ) ;
#75048=ORIENTED_EDGE ( 'NONE', *, *, #60760, .F. ) ;
#75049=EDGE_LOOP ( 'NONE', ( #89114, #80942, #75911, #93948 ) ) ;
#75050=ORIENTED_EDGE ( 'NONE', *, *, #58369, .T. ) ;
#75051=DIRECTION ( 'NONE',  ( 0.000000000000000000, 0.000000000000000000, 1.000000000000000000 ) ) ;
#75052=CARTESIAN_POINT ( 'NONE',  ( -4.600000000000025402, 2.500000000000000000, -2.385244779468109755E-15 ) ) ;
#75053=LINE ( 'NONE', #25956, #94805 ) ;
#75054=CONICAL_SURFACE ( 'NONE', #98029, 0.09999999999999982514, 0.003490658503988666988 ) ;
#75055=ORIENTED_EDGE ( 'NONE', *, *, #9351, .T. ) ;
#75056=CARTESIAN_POINT ( 'NONE',  ( 3.710216157319381924, 2.500000000002297718, -9.999999999875349488 ) ) ;
#75057=DIRECTION ( 'NONE',  ( 0.000000000000000000, -0.9999939076577903929, 0.003490651415223739937 ) ) ;
#75058=DIRECTION ( 'NONE',  ( -0.000000000000000000, -1.000000000000000000, -0.000000000000000000 ) ) ;
#75059=AXIS2_PLACEMENT_3D ( 'NONE', #71960, #2540, #51035 ) ;
#75061=DIRECTION ( 'NONE',  ( 0.000000000000000000, 1.000000000000000000, 0.000000000000000000 ) ) ;
#75062=AXIS2_PLACEMENT_3D ( 'NONE', #99195, #31736, #11444 ) ;
#75063=DIRECTION ( 'NONE',  ( 0.000000000000000000, -0.000000000000000000, 1.000000000000000000 ) ) ;
#75064=EDGE_LOOP ( 'NONE', ( #70106, #47564 ) ) ;
#75065=CARTESIAN_POINT ( 'NONE',  ( -2.499999999999996447, 2.500000000000000000, 4.430127018922196847 ) ) ;
#75066=AXIS2_PLACEMENT_3D ( 'NONE', #82367, #122286, #32639 ) ;
#75067=AXIS2_PLACEMENT_3D ( 'NONE', #92698, #32514, #112341 ) ;
#75070=DIRECTION ( 'NONE',  ( 0.000000000000000000, 1.000000000000000000, 0.000000000000000000 ) ) ;
#75071=DIRECTION ( 'NONE',  ( 0.000000000000000000, 0.000000000000000000, -1.000000000000000000 ) ) ;
#75072=DIRECTION ( 'NONE',  ( 0.000000000000000000, -0.9999939076577903929, 0.003490651415223739937 ) ) ;
#75073=CARTESIAN_POINT ( 'NONE',  ( 13.54999999999989946, 12.50000000000000000, 2.511473670974873507 ) ) ;
#75074=CARTESIAN_POINT ( 'NONE',  ( 3.149999999999944400, 2.500000000000000000, 2.511473670974873507 ) ) ;
#75075=ORIENTED_EDGE ( 'NONE', *, *, #8992, .F. ) ;
#75076=VERTEX_POINT ( 'NONE', #83176 ) ;
#75077=EDGE_CURVE ( 'NONE', #70759, #49015, #127166, .T. ) ;
#75079=DIRECTION ( 'NONE',  ( 0.000000000000000000, 0.000000000000000000, -1.000000000000000000 ) ) ;
#75080=PLANE ( 'NONE',  #121300 ) ;
#75081=AXIS2_PLACEMENT_3D ( 'NONE', #17544, #76491, #35910 ) ;
#75082=ORIENTED_EDGE ( 'NONE', *, *, #17978, .F. ) ;
#75084=DIRECTION ( 'NONE',  ( -4.274815082592931898E-19, -0.9999939076577903929, -0.003490651415223739937 ) ) ;
#75085=VERTEX_POINT ( 'NONE', #63533 ) ;
#75086=CARTESIAN_POINT ( 'NONE',  ( -1.650000000000034772, 2.500000000000000000, 1.372243186433545370 ) ) ;
#75087=CIRCLE ( 'NONE', #64615, 0.06509327318403745899 ) ;
#75088=AXIS2_PLACEMENT_3D ( 'NONE', #107299, #107953, #89601 ) ;
#75089=DIRECTION ( 'NONE',  ( 0.000000000000000000, 1.000000000000000000, 0.000000000000000000 ) ) ;
#75090=ORIENTED_EDGE ( 'NONE', *, *, #29787, .T. ) ;
#75091=PLANE ( 'NONE',  #127597 ) ;
#75092=DIRECTION ( 'NONE',  ( -4.274815082592931898E-19, -0.9999939076577903929, -0.003490651415223739937 ) ) ;
#75093=FACE_OUTER_BOUND ( 'NONE', #39009, .T. ) ;
#75094=ADVANCED_FACE ( 'NONE', ( #73331 ), #42617, .T. ) ;
#75095=EDGE_CURVE ( 'NONE', #34711, #105977, #125005, .T. ) ;
#75096=DIRECTION ( 'NONE',  ( 0.000000000000000000, 0.000000000000000000, 1.000000000000000000 ) ) ;
#75097=AXIS2_PLACEMENT_3D ( 'NONE', #4745, #2183, #44706 ) ;
#75099=AXIS2_PLACEMENT_3D ( 'NONE', #95380, #5691, #72531 ) ;
#75100=CIRCLE ( 'NONE', #91827, 0.1000000000000002554 ) ;
#75101=DIRECTION ( 'NONE',  ( -0.000000000000000000, -1.000000000000000000, -0.000000000000000000 ) ) ;
#75102=DIRECTION ( 'NONE',  ( -4.274815082592931898E-19, -0.9999939076577903929, -0.003490651415223739937 ) ) ;
#75103=EDGE_LOOP ( 'NONE', ( #124424, #109074 ) ) ;
#75104=ORIENTED_EDGE ( 'NONE', *, *, #106281, .T. ) ;
#75105=EDGE_CURVE ( 'NONE', #10740, #65870, #87430, .T. ) ;
#75106=FACE_OUTER_BOUND ( 'NONE', #124771, .T. ) ;
#75107=CARTESIAN_POINT ( 'NONE',  ( 12.49999999999990230, 2.500000000000000000, -0.6928203230275541413 ) ) ;
#75108=FACE_OUTER_BOUND ( 'NONE', #59083, .T. ) ;
#75109=AXIS2_PLACEMENT_3D ( 'NONE', #92551, #19957, #101738 ) ;
#75110=CARTESIAN_POINT ( 'NONE',  ( 4.349999999999940137, 12.50000000000000000, -2.511473670974877948 ) ) ;
#75111=CARTESIAN_POINT ( 'NONE',  ( -5.400000000000024336, 12.50000000000000000, -3.637306695894650055 ) ) ;
#75112=VECTOR ( 'NONE', #107961, 1000.000000000000000 ) ;
#75113=DIRECTION ( 'NONE',  ( -0.000000000000000000, 1.000000000000000000, -0.000000000000000000 ) ) ;
#75114=DIRECTION ( 'NONE',  ( -0.000000000000000000, 1.000000000000000000, -0.000000000000000000 ) ) ;
#75115=LINE ( 'NONE', #25347, #89611 ) ;
#75116=CARTESIAN_POINT ( 'NONE',  ( -7.100000000000017408, 2.500000000000000000, -0.6928203230275542523 ) ) ;
#75117=DIRECTION ( 'NONE',  ( -0.000000000000000000, -1.000000000000000000, -0.000000000000000000 ) ) ;
#75119=EDGE_LOOP ( 'NONE', ( #79036, #114272 ) ) ;
#75120=CONICAL_SURFACE ( 'NONE', #18681, 0.1000000000000000472, 0.003490658503988666988 ) ;
#75121=ORIENTED_EDGE ( 'NONE', *, *, #19557, .F. ) ;
#75122=DIRECTION ( 'NONE',  ( -0.000000000000000000, 1.000000000000000000, -0.000000000000000000 ) ) ;
#75123=CARTESIAN_POINT ( 'NONE',  ( 7.499999999999927169, 12.50000000000000000, 3.637306695894644726 ) ) ;
#75124=CARTESIAN_POINT ( 'NONE',  ( -7.700000000000014388, 2.500000000000000000, -0.3464101615137782364 ) ) ;
#75125=ORIENTED_EDGE ( 'NONE', *, *, #46021, .F. ) ;
#75126=CARTESIAN_POINT ( 'NONE',  ( 3.749999999999944045, 2.500000000000000000, -2.957883832488653830 ) ) ;
#75127=EDGE_CURVE ( 'NONE', #4337, #39809, #2648, .T. ) ;
#75128=CARTESIAN_POINT ( 'NONE',  ( 11.04999999999991189, 2.500000000000000000, 6.148780366869520897 ) ) ;
#75129=DIRECTION ( 'NONE',  ( 0.000000000000000000, -0.000000000000000000, 1.000000000000000000 ) ) ;
#75130=ORIENTED_EDGE ( 'NONE', *, *, #6534, .T. ) ;
#75131=EDGE_CURVE ( 'NONE', #97166, #74962, #22961, .T. ) ;
#75132=AXIS2_PLACEMENT_3D ( 'NONE', #23749, #32941, #53846 ) ;
#75133=EDGE_CURVE ( 'NONE', #47787, #67958, #28874, .T. ) ;
#75134=CARTESIAN_POINT ( 'NONE',  ( -3.100000000000028955, 12.50000000000000000, 4.676537180435972552 ) ) ;
#75135=ORIENTED_EDGE ( 'NONE', *, *, #57739, .F. ) ;
#75136=VERTEX_POINT ( 'NONE', #34073 ) ;
#75137=EDGE_LOOP ( 'NONE', ( #102499, #4678, #22483, #54454 ) ) ;
#75138=EDGE_LOOP ( 'NONE', ( #47555, #77519, #41605, #103237 ) ) ;
#75139=DIRECTION ( 'NONE',  ( 0.000000000000000000, 1.000000000000000000, 0.000000000000000000 ) ) ;
#75140=ADVANCED_FACE ( 'NONE', ( #13763 ), #24752, .T. ) ;
#75141=EDGE_CURVE ( 'NONE', #64674, #5452, #81190, .T. ) ;
#75142=CIRCLE ( 'NONE', #123262, 0.1000000000000000472 ) ;
#75143=ADVANCED_FACE ( 'NONE', ( #112632 ), #123046, .T. ) ;
#75144=EDGE_CURVE ( 'NONE', #81046, #107875, #102163, .T. ) ;
#75145=DIRECTION ( 'NONE',  ( -0.000000000000000000, -1.000000000000000000, -0.000000000000000000 ) ) ;
#75146=PLANE ( 'NONE',  #88050 ) ;
#75147=CARTESIAN_POINT ( 'NONE',  ( -12.69999999999999218, 12.50000000000000000, 4.676537180435972552 ) ) ;
#75148=ORIENTED_EDGE ( 'NONE', *, *, #112374, .T. ) ;
#75149=CONICAL_SURFACE ( 'NONE', #60502, 0.1000000000000000472, 0.003490658503988666988 ) ;
#75150=CONICAL_SURFACE ( 'NONE', #16635, 0.09999999999999982514, 0.003490658503988666988 ) ;
#75151=ADVANCED_FACE ( 'NONE', ( #13111 ), #54087, .T. ) ;
#75152=DIRECTION ( 'NONE',  ( -0.000000000000000000, -1.000000000000000000, -0.000000000000000000 ) ) ;
#75153=ORIENTED_EDGE ( 'NONE', *, *, #54873, .F. ) ;
#75154=CARTESIAN_POINT ( 'NONE',  ( 3.549999999999943867, 2.500000000000000000, -6.048780366869526581 ) ) ;
#75155=CARTESIAN_POINT ( 'NONE',  ( 9.549999999999918998, 12.50000000000000000, -6.495190528383302464 ) ) ;
#75156=VECTOR ( 'NONE', #116088, 1000.000000000000000 ) ;
#75157=DIRECTION ( 'NONE',  ( 0.000000000000000000, 1.000000000000000000, 0.000000000000000000 ) ) ;
#75158=CARTESIAN_POINT ( 'NONE',  ( 18.98912670146762594, -2.543039972613341693, 4.488908218019908247 ) ) ;
#75159=EDGE_CURVE ( 'NONE', #42013, #54592, #95856, .T. ) ;
#75160=ORIENTED_EDGE ( 'NONE', *, *, #103331, .F. ) ;
#75161=CONICAL_SURFACE ( 'NONE', #89816, 0.1000000000000002554, 0.003490658503988666988 ) ;
#75162=AXIS2_PLACEMENT_3D ( 'NONE', #16046, #55981, #95914 ) ;
#75163=ORIENTED_EDGE ( 'NONE', *, *, #43119, .F. ) ;
#75164=EDGE_LOOP ( 'NONE', ( #75480, #116932, #73696, #93400, #26448 ) ) ;
#75165=DIRECTION ( 'NONE',  ( 0.000000000000000000, 0.000000000000000000, -1.000000000000000000 ) ) ;
#75166=CARTESIAN_POINT ( 'NONE',  ( -3.350000000000028511, 12.50000000000000000, -2.857883832488653741 ) ) ;
#75167=DIRECTION ( 'NONE',  ( -0.000000000000000000, 1.000000000000000000, -0.000000000000000000 ) ) ;
#75168=FACE_BOUND ( 'NONE', #26828, .T. ) ;
#75169=CARTESIAN_POINT ( 'NONE',  ( 5.849999999999933031, 12.50000000000000000, 7.253104124594885960 ) ) ;
#75170=CARTESIAN_POINT ( 'NONE',  ( 6.849999999999927702, 12.50000000000000000, 2.576566944158910744 ) ) ;
#75171=DIRECTION ( 'NONE',  ( 0.000000000000000000, 0.000000000000000000, 1.000000000000000000 ) ) ;
#75172=LINE ( 'NONE', #95459, #123692 ) ;
#75173=DIRECTION ( 'NONE',  ( 0.000000000000000000, 0.000000000000000000, 1.000000000000000000 ) ) ;
#75175=ORIENTED_EDGE ( 'NONE', *, *, #113084, .T. ) ;
#75176=AXIS2_PLACEMENT_3D ( 'NONE', #29118, #50668, #59876 ) ;
#75177=AXIS2_PLACEMENT_3D ( 'NONE', #24728, #23430, #63366 ) ;
#75178=CARTESIAN_POINT ( 'NONE',  ( -13.94999999999998685, 12.50000000000000000, 1.818653347947325472 ) ) ;
#75179=EDGE_LOOP ( 'NONE', ( #103335, #27757 ) ) ;
#75180=EDGE_LOOP ( 'NONE', ( #123117, #119512, #112768, #66530 ) ) ;
#75181=ORIENTED_EDGE ( 'NONE', *, *, #21714, .F. ) ;
#75182=ORIENTED_EDGE ( 'NONE', *, *, #65735, .F. ) ;
#75183=DIRECTION ( 'NONE',  ( 0.000000000000000000, -0.9999939076577903929, 0.003490651415223739937 ) ) ;
#75184=FACE_BOUND ( 'NONE', #77906, .T. ) ;
#75185=CARTESIAN_POINT ( 'NONE',  ( -1.850000000000033840, 2.500000000000000000, 1.818653347947321475 ) ) ;
#75186=CONICAL_SURFACE ( 'NONE', #100231, 0.1000000000000000472, 0.003490658503988666988 ) ;
#75187=CONICAL_SURFACE ( 'NONE', #29234, 0.1000000000000002554, 0.003490658503988666988 ) ;
#75188=AXIS2_PLACEMENT_3D ( 'NONE', #1339, #48518, #28887 ) ;
#75189=ADVANCED_FACE ( 'NONE', ( #121153 ), #114719, .T. ) ;
#75190=ORIENTED_EDGE ( 'NONE', *, *, #35060, .F. ) ;
#75191=CARTESIAN_POINT ( 'NONE',  ( 87.49999999944498086, 3.974992050012154277, 6.359987280019447020 ) ) ;
#75192=DIRECTION ( 'NONE',  ( 0.000000000000000000, 0.000000000000000000, -1.000000000000000000 ) ) ;
#75193=CONICAL_SURFACE ( 'NONE', #125366, 0.1000000000000002554, 0.003490658503988666988 ) ;
#75194=VERTEX_POINT ( 'NONE', #52410 ) ;
#75195=CARTESIAN_POINT ( 'NONE',  ( 8.149999999999923972, 12.50000000000000000, -6.148780366869526226 ) ) ;
#75196=CARTESIAN_POINT ( 'NONE',  ( -5.400000000000019895, 2.500000000000000000, 3.637306695894644726 ) ) ;
#75197=ADVANCED_FACE ( 'NONE', ( #21674 ), #58305, .T. ) ;
#75198=CIRCLE ( 'NONE', #119023, 0.09999999999999999167 ) ;
#75199=AXIS2_PLACEMENT_3D ( 'NONE', #83374, #5435, #84655 ) ;
#75200=ORIENTED_EDGE ( 'NONE', *, *, #102176, .F. ) ;
#75201=DIRECTION ( 'NONE',  ( 0.000000000000000000, 0.000000000000000000, 1.000000000000000000 ) ) ;
#75203=CONICAL_SURFACE ( 'NONE', #18765, 0.1000000000000002554, 0.003490658503988666988 ) ;
#75204=VERTEX_POINT ( 'NONE', #11833 ) ;
#75205=DIRECTION ( 'NONE',  ( -0.000000000000000000, 1.000000000000000000, -0.000000000000000000 ) ) ;
#75206=CARTESIAN_POINT ( 'NONE',  ( -0.8500000000000390576, 2.500000000000000000, -6.495190528383302464 ) ) ;
#75207=CARTESIAN_POINT ( 'NONE',  ( 2.699999999999947331, 12.50000000000000000, -0.4115034346978157509 ) ) ;
#75208=VECTOR ( 'NONE', #60443, 1000.000000000000000 ) ;
#75209=ORIENTED_EDGE ( 'NONE', *, *, #56897, .F. ) ;
#75210=ORIENTED_EDGE ( 'NONE', *, *, #30560, .T. ) ;
#75211=DIRECTION ( 'NONE',  ( -4.274815082592931898E-19, -0.9999939076577903929, -0.003490651415223739937 ) ) ;
#75212=ORIENTED_EDGE ( 'NONE', *, *, #32226, .F. ) ;
#75213=FACE_OUTER_BOUND ( 'NONE', #11502, .T. ) ;
#75214=DIRECTION ( 'NONE',  ( 0.000000000000000000, 0.000000000000000000, 1.000000000000000000 ) ) ;
#75215=ORIENTED_EDGE ( 'NONE', *, *, #64067, .T. ) ;
#75217=DIRECTION ( 'NONE',  ( -0.000000000000000000, -1.000000000000000000, -0.000000000000000000 ) ) ;
#75218=DIRECTION ( 'NONE',  ( 0.000000000000000000, -0.9999939076577903929, 0.003490651415223739937 ) ) ;
#75219=CARTESIAN_POINT ( 'NONE',  ( -5.600000000000023626, 12.50000000000000000, -3.983716857408426293 ) ) ;
#75220=DIRECTION ( 'NONE',  ( 0.000000000000000000, -0.9999939076577903929, 0.003490651415223739937 ) ) ;
#75221=ORIENTED_EDGE ( 'NONE', *, *, #52997, .T. ) ;
#75222=EDGE_CURVE ( 'NONE', #179, #49864, #102115, .T. ) ;
#75223=EDGE_LOOP ( 'NONE', ( #86012, #60031 ) ) ;
#75224=PLANE ( 'NONE',  #18155 ) ;
#75225=CARTESIAN_POINT ( 'NONE',  ( 17.91370874550463554, -0.4812889678259977266, 4.985910759330125508 ) ) ;
#75226=DIRECTION ( 'NONE',  ( 0.000000000000000000, 0.000000000000000000, -1.000000000000000000 ) ) ;
#75227=ORIENTED_EDGE ( 'NONE', *, *, #72783, .F. ) ;
#75228=EDGE_LOOP ( 'NONE', ( #35958, #129358, #1325, #68419 ) ) ;
#75229=VERTEX_POINT ( 'NONE', #81859 ) ;
#75230=AXIS2_PLACEMENT_3D ( 'NONE', #49013, #9717, #49660 ) ;
#75231=DIRECTION ( 'NONE',  ( -0.000000000000000000, -1.000000000000000000, -0.000000000000000000 ) ) ;
#75232=CARTESIAN_POINT ( 'NONE',  ( -5.850000000000018296, 2.500000000000000000, 1.472243186433545459 ) ) ;
#75233=ADVANCED_FACE ( 'NONE', ( #62249 ), #76571, .T. ) ;
#75234=CARTESIAN_POINT ( 'NONE',  ( 5.849999999999933920, 12.50000000000000000, 5.802370205355744659 ) ) ;
#75235=AXIS2_PLACEMENT_3D ( 'NONE', #69006, #95899, #67714 ) ;
#75236=AXIS2_PLACEMENT_3D ( 'NONE', #125403, #75636, #45566 ) ;
#75237=DIRECTION ( 'NONE',  ( 0.000000000000000000, 0.000000000000000000, 1.000000000000000000 ) ) ;
#75238=CARTESIAN_POINT ( 'NONE',  ( -3.150000000000030553, 12.50000000000000000, 6.213873640053558134 ) ) ;
#75239=CARTESIAN_POINT ( 'NONE',  ( -5.650000000000019895, 2.500000000000000000, 2.611473670974873151 ) ) ;
#75240=FACE_OUTER_BOUND ( 'NONE', #120591, .T. ) ;
#75241=CARTESIAN_POINT ( 'NONE',  ( -3.150000000000029665, 12.50000000000000000, 6.841600689897072485 ) ) ;
#75242=EDGE_CURVE ( 'NONE', #116514, #109859, #74629, .T. ) ;
#75243=ADVANCED_FACE ( 'NONE', ( #26184 ), #36664, .T. ) ;
#75244=CARTESIAN_POINT ( 'NONE',  ( -5.200000000000020606, 2.500000000000000000, -0.4464101615137782142 ) ) ;
#75245=CIRCLE ( 'NONE', #91973, 0.1000000000000002554 ) ;
#75246=CONICAL_SURFACE ( 'NONE', #79184, 0.1000000000000000472, 0.003490658503988666988 ) ;
#75247=VERTEX_POINT ( 'NONE', #15692 ) ;
#75248=ADVANCED_FACE ( 'NONE', ( #86375 ), #112587, .T. ) ;
#75249=DIRECTION ( 'NONE',  ( -4.274815082592931898E-19, -0.9999939076577903929, -0.003490651415223739937 ) ) ;
#75250=VERTEX_POINT ( 'NONE', #16330 ) ;
#75251=ORIENTED_EDGE ( 'NONE', *, *, #98158, .T. ) ;
#75252=ADVANCED_FACE ( 'NONE', ( #114542 ), #41593, .T. ) ;
#75253=CARTESIAN_POINT ( 'NONE',  ( 7.899999999999924860, 12.50000000000000000, -3.637306695894650055 ) ) ;
#75254=CARTESIAN_POINT ( 'NONE',  ( 4.399999999999937295, 2.500000000000000000, 4.083716857408421497 ) ) ;
#75255=DIRECTION ( 'NONE',  ( 0.000000000000000000, 1.000000000000000000, 0.000000000000000000 ) ) ;
#75256=DIRECTION ( 'NONE',  ( 0.000000000000000000, 1.000000000000000000, 0.000000000000000000 ) ) ;
#75257=CARTESIAN_POINT ( 'NONE',  ( 5.399999999999932854, 2.500000000000000000, 5.022947341949748790 ) ) ;
#75258=DIRECTION ( 'NONE',  ( 0.000000000000000000, -0.9999939076577903929, 0.003490651415223739937 ) ) ;
#75259=ORIENTED_EDGE ( 'NONE', *, *, #106176, .T. ) ;
#75261=CARTESIAN_POINT ( 'NONE',  ( 4.599999999999935696, 2.500000000000000000, 4.922947341949748257 ) ) ;
#75262=EDGE_LOOP ( 'NONE', ( #100882, #42307 ) ) ;
#75263=AXIS2_PLACEMENT_3D ( 'NONE', #105994, #56867, #117720 ) ;
#75264=CONICAL_SURFACE ( 'NONE', #52291, 0.1000000000000002554, 0.003490658503988666988 ) ;
#75265=ORIENTED_EDGE ( 'NONE', *, *, #50132, .T. ) ;
#75266=ORIENTED_EDGE ( 'NONE', *, *, #31336, .T. ) ;
#75267=EDGE_LOOP ( 'NONE', ( #93111, #102870 ) ) ;
#75268=DIRECTION ( 'NONE',  ( -0.000000000000000000, -1.000000000000000000, -0.000000000000000000 ) ) ;
#75269=CARTESIAN_POINT ( 'NONE',  ( 7.299999999999924327, 2.500000000000000000, 0.4464101615137735513 ) ) ;
#75270=CIRCLE ( 'NONE', #18835, 0.06509327318403743123 ) ;
#75271=CARTESIAN_POINT ( 'NONE',  ( -3.150000000000029221, 12.50000000000000000, -1.818653347947326138 ) ) ;
#75272=CARTESIAN_POINT ( 'NONE',  ( 5.399999999999936406, 12.50000000000000000, -4.957854068765716882 ) ) ;
#75273=CARTESIAN_POINT ( 'NONE',  ( -4.800000000000024691, 2.500000000000000000, 0.2464101615137735679 ) ) ;
#75274=EDGE_LOOP ( 'NONE', ( #5359, #38401 ) ) ;
#75275=CARTESIAN_POINT ( 'NONE',  ( 11.04999999999990834, 2.500000000000000000, -6.841600689897077814 ) ) ;
#75276=CARTESIAN_POINT ( 'NONE',  ( -4.200000000000029488, 12.50000000000000000, -4.330127018922201643 ) ) ;
#75277=AXIS2_PLACEMENT_3D ( 'NONE', #3375, #52469, #104157 ) ;
#75278=ADVANCED_FACE ( 'NONE', ( #124387 ), #77070, .T. ) ;
#75279=CARTESIAN_POINT ( 'NONE',  ( 6.049999999999932321, 2.500000000000000000, -1.818653347947326138 ) ) ;
#75280=CIRCLE ( 'NONE', #29248, 0.06509327318403745899 ) ;
#75281=ORIENTED_EDGE ( 'NONE', *, *, #85632, .T. ) ;
#75282=AXIS2_PLACEMENT_3D ( 'NONE', #14448, #45874, #75959 ) ;
#75283=ORIENTED_EDGE ( 'NONE', *, *, #123069, .T. ) ;
#75284=ORIENTED_EDGE ( 'NONE', *, *, #49073, .F. ) ;
#75285=EDGE_CURVE ( 'NONE', #69514, #4494, #51953, .T. ) ;
#75286=DIRECTION ( 'NONE',  ( 0.000000000000000000, 1.000000000000000000, 0.000000000000000000 ) ) ;
#75287=EDGE_CURVE ( 'NONE', #88053, #60113, #110521, .T. ) ;
#75288=EDGE_CURVE ( 'NONE', #51687, #33188, #125092, .T. ) ;
#75289=CIRCLE ( 'NONE', #21004, 0.1000000000000000472 ) ;
#75290=ADVANCED_FACE ( 'NONE', ( #36006 ), #96837, .T. ) ;
#75291=CARTESIAN_POINT ( 'NONE',  ( 2.949999999999946887, 2.500000000000000000, -2.265063509461101798 ) ) ;
#75292=FACE_OUTER_BOUND ( 'NONE', #123983, .T. ) ;
#75293=EDGE_CURVE ( 'NONE', #17445, #32739, #85386, .T. ) ;
#75294=ORIENTED_EDGE ( 'NONE', *, *, #40414, .T. ) ;
#75295=CARTESIAN_POINT ( 'NONE',  ( 13.94999999999989271, 12.50000000000000000, -1.818653347947326138 ) ) ;
#75296=DIRECTION ( 'NONE',  ( -0.000000000000000000, -1.000000000000000000, -0.000000000000000000 ) ) ;
#75297=CARTESIAN_POINT ( 'NONE',  ( -7.900000000000011013, 12.50000000000000000, 4.330127018922196314 ) ) ;
#75298=CARTESIAN_POINT ( 'NONE',  ( 10.64999999999991331, 2.500000000000000000, 6.248780366869521430 ) ) ;
#75299=DIRECTION ( 'NONE',  ( 0.000000000000000000, 1.000000000000000000, 0.000000000000000000 ) ) ;
#75300=ADVANCED_FACE ( 'NONE', ( #45827 ), #49897, .T. ) ;
#75301=ORIENTED_EDGE ( 'NONE', *, *, #18225, .F. ) ;
#75302=EDGE_CURVE ( 'NONE', #83089, #85131, #104264, .T. ) ;
#75303=CARTESIAN_POINT ( 'NONE',  ( 13.14999999999989733, 12.50000000000000000, -2.511473670974877948 ) ) ;
#75304=EDGE_LOOP ( 'NONE', ( #120223, #1264, #112826, #4994 ) ) ;
#75305=ORIENTED_EDGE ( 'NONE', *, *, #122529, .T. ) ;
#75306=ORIENTED_EDGE ( 'NONE', *, *, #28265, .T. ) ;
#75307=CARTESIAN_POINT ( 'NONE',  ( -3.750000000000027978, 12.50000000000000000, 7.188010851410848723 ) ) ;
#75308=FACE_BOUND ( 'NONE', #122071, .T. ) ;
#75309=CARTESIAN_POINT ( 'NONE',  ( -3.350000000000031619, 2.500000000000000000, -5.902370205355750521 ) ) ;
#75310=DIRECTION ( 'NONE',  ( 0.000000000000000000, -0.9999939076577903929, 0.003490651415223739937 ) ) ;
#75311=CARTESIAN_POINT ( 'NONE',  ( 5.399999999999932854, 2.500000000000000000, 5.022947341949748790 ) ) ;
#75312=AXIS2_PLACEMENT_3D ( 'NONE', #122738, #52706, #112917 ) ;
#75313=ORIENTED_EDGE ( 'NONE', *, *, #124002, .F. ) ;
#75314=CARTESIAN_POINT ( 'NONE',  ( 14.99999999999989342, 2.500000000000000000, -0.6928203230275541413 ) ) ;
#75315=VECTOR ( 'NONE', #56067, 1000.000000000000000 ) ;
#75316=CARTESIAN_POINT ( 'NONE',  ( 9.199999999999919353, 2.500000000000000000, -2.276824562219559311E-15 ) ) ;
#75317=DIRECTION ( 'NONE',  ( 0.000000000000000000, 1.000000000000000000, 0.000000000000000000 ) ) ;
#75318=FACE_OUTER_BOUND ( 'NONE', #28980, .T. ) ;
#75319=EDGE_LOOP ( 'NONE', ( #41436, #106951, #44515, #71621 ) ) ;
#75320=CARTESIAN_POINT ( 'NONE',  ( 1.649999999999948841, 12.50000000000000000, 6.560283801567334372 ) ) ;
#75321=CIRCLE ( 'NONE', #58617, 0.06509327318403745899 ) ;
#75322=VECTOR ( 'NONE', #14620, 1000.000000000000000 ) ;
#75323=CARTESIAN_POINT ( 'NONE',  ( 4.399999999999939071, 2.500000000000000000, -0.3464101615137782364 ) ) ;
#75324=ORIENTED_EDGE ( 'NONE', *, *, #100441, .T. ) ;
#75325=FACE_OUTER_BOUND ( 'NONE', #121271, .T. ) ;
#75326=EDGE_LOOP ( 'NONE', ( #89466, #1636, #123878, #68259 ) ) ;
#75327=FACE_BOUND ( 'NONE', #64427, .T. ) ;
#75328=DIRECTION ( 'NONE',  ( 0.000000000000000000, 1.000000000000000000, 0.000000000000000000 ) ) ;
#75329=ORIENTED_EDGE ( 'NONE', *, *, #74826, .F. ) ;
#75330=DIRECTION ( 'NONE',  ( 0.000000000000000000, 0.000000000000000000, 1.000000000000000000 ) ) ;
#75331=DIRECTION ( 'NONE',  ( 0.000000000000000000, 0.000000000000000000, 1.000000000000000000 ) ) ;
#75332=EDGE_LOOP ( 'NONE', ( #33130, #50782 ) ) ;
#75333=ORIENTED_EDGE ( 'NONE', *, *, #60039, .T. ) ;
#75335=ORIENTED_EDGE ( 'NONE', *, *, #93458, .F. ) ;
#75337=DIRECTION ( 'NONE',  ( -0.000000000000000000, -1.000000000000000000, -0.000000000000000000 ) ) ;
#75338=EDGE_CURVE ( 'NONE', #87541, #105417, #62422, .T. ) ;
#75339=CARTESIAN_POINT ( 'NONE',  ( -13.29999999999999005, 2.500000000000000000, -4.330127018922198978 ) ) ;
#75340=DIRECTION ( 'NONE',  ( -0.000000000000000000, -1.000000000000000000, -0.000000000000000000 ) ) ;
#75341=CARTESIAN_POINT ( 'NONE',  ( -2.500000000000032419, 2.500000000000000000, 0.6928203230275494784 ) ) ;
#75342=CARTESIAN_POINT ( 'NONE',  ( -10.84999999999999964, 12.50000000000000000, 1.537336459617582918 ) ) ;
#75343=AXIS2_PLACEMENT_3D ( 'NONE', #9912, #1366, #121151 ) ;
#75344=EDGE_LOOP ( 'NONE', ( #49261, #107030, #17784, #47853 ) ) ;
#75345=ORIENTED_EDGE ( 'NONE', *, *, #56473, .T. ) ;
#75346=DIRECTION ( 'NONE',  ( 0.000000000000000000, 0.000000000000000000, -1.000000000000000000 ) ) ;
#75347=CARTESIAN_POINT ( 'NONE',  ( 8.149999999999923972, 2.500000000000000000, -6.248780366869526759 ) ) ;
#75348=CARTESIAN_POINT ( 'NONE',  ( 10.39999999999991331, 2.500000000000000000, -2.385244779468109755E-15 ) ) ;
#75350=ORIENTED_EDGE ( 'NONE', *, *, #35282, .T. ) ;
#75351=VERTEX_POINT ( 'NONE', #75269 ) ;
#75352=FACE_BOUND ( 'NONE', #12903, .T. ) ;
#75353=EDGE_LOOP ( 'NONE', ( #22054, #44707, #20060, #72717, #116026, #18415 ) ) ;
#75354=CARTESIAN_POINT ( 'NONE',  ( -10.20000000000000462, 12.50000000000000000, -4.611443907251935315 ) ) ;
#75355=CARTESIAN_POINT ( 'NONE',  ( 11.89999999999990798, 12.50000000000000000, -4.676537180435977881 ) ) ;
#75356=AXIS2_PLACEMENT_3D ( 'NONE', #89478, #51501, #91407 ) ;
#75357=ORIENTED_EDGE ( 'NONE', *, *, #85798, .T. ) ;
#75358=DIRECTION ( 'NONE',  ( 0.000000000000000000, 1.000000000000000000, 0.000000000000000000 ) ) ;
#75359=FACE_OUTER_BOUND ( 'NONE', #102422, .T. ) ;
#75360=DIRECTION ( 'NONE',  ( 0.000000000000000000, 0.000000000000000000, 1.000000000000000000 ) ) ;
#75361=DIRECTION ( 'NONE',  ( 0.000000000000000000, 1.000000000000000000, 0.000000000000000000 ) ) ;
#75363=DIRECTION ( 'NONE',  ( 0.000000000000000000, 0.000000000000000000, 1.000000000000000000 ) ) ;
#75365=FACE_OUTER_BOUND ( 'NONE', #105822, .T. ) ;
#75366=FACE_OUTER_BOUND ( 'NONE', #16211, .T. ) ;
#75367=EDGE_LOOP ( 'NONE', ( #109045, #114028, #19689, #83813 ) ) ;
#75368=AXIS2_PLACEMENT_3D ( 'NONE', #84335, #54237, #94152 ) ;
#75369=ORIENTED_EDGE ( 'NONE', *, *, #53430, .F. ) ;
#75370=DIRECTION ( 'NONE',  ( 0.000000000000000000, 0.000000000000000000, -1.000000000000000000 ) ) ;
#75371=EDGE_LOOP ( 'NONE', ( #100784, #68853 ) ) ;
#75372=LINE ( 'NONE', #35474, #1833 ) ;
#75373=EDGE_LOOP ( 'NONE', ( #18528, #113343 ) ) ;
#75374=VERTEX_POINT ( 'NONE', #73990 ) ;
#75376=FACE_OUTER_BOUND ( 'NONE', #48898, .T. ) ;
#75377=AXIS2_PLACEMENT_3D ( 'NONE', #14293, #63413, #51672 ) ;
#75378=EDGE_CURVE ( 'NONE', #100973, #115124, #113923, .T. ) ;
#75379=DIRECTION ( 'NONE',  ( 0.000000000000000000, 1.000000000000000000, 0.000000000000000000 ) ) ;
#75380=CARTESIAN_POINT ( 'NONE',  ( -13.54999999999998828, 2.500000000000000000, 1.718653347947325383 ) ) ;
#75381=AXIS2_PLACEMENT_3D ( 'NONE', #102069, #12387, #2549 ) ;
#75382=FACE_OUTER_BOUND ( 'NONE', #103259, .T. ) ;
#75383=DIRECTION ( 'NONE',  ( 0.000000000000000000, 1.000000000000000000, 0.000000000000000000 ) ) ;
#75384=EDGE_CURVE ( 'NONE', #32532, #40814, #87519, .T. ) ;
#75385=EDGE_LOOP ( 'NONE', ( #122069, #19637, #45922, #56020 ) ) ;
#75386=ADVANCED_FACE ( 'NONE', ( #35363 ), #125019, .T. ) ;
#75387=DIRECTION ( 'NONE',  ( -0.000000000000000000, 1.000000000000000000, -0.000000000000000000 ) ) ;
#75388=ORIENTED_EDGE ( 'NONE', *, *, #101281, .T. ) ;
#75389=ORIENTED_EDGE ( 'NONE', *, *, #114716, .T. ) ;
#75390=ORIENTED_EDGE ( 'NONE', *, *, #105946, .F. ) ;
#75391=ORIENTED_EDGE ( 'NONE', *, *, #107367, .T. ) ;
#75392=ADVANCED_FACE ( 'NONE', ( #37931 ), #27447, .T. ) ;
#75393=DIRECTION ( 'NONE',  ( -0.000000000000000000, 1.000000000000000000, -0.000000000000000000 ) ) ;
#75394=EDGE_CURVE ( 'NONE', #97846, #51736, #119704, .T. ) ;
#75396=ADVANCED_FACE ( 'NONE', ( #50331 ), #18918, .T. ) ;
#75397=VERTEX_POINT ( 'NONE', #20228 ) ;
#75398=ORIENTED_EDGE ( 'NONE', *, *, #41866, .T. ) ;
#75399=ADVANCED_FACE ( 'NONE', ( #58861 ), #91644, .T. ) ;
#75400=CARTESIAN_POINT ( 'NONE',  ( 2.099999999999948574, 12.50000000000000000, 3.702399969078682407 ) ) ;
#75401=CARTESIAN_POINT ( 'NONE',  ( 6.049999999999932321, 2.500000000000000000, 6.841600689897072485 ) ) ;
#75402=DIRECTION ( 'NONE',  ( 0.000000000000000000, 0.000000000000000000, 1.000000000000000000 ) ) ;
#75403=DIRECTION ( 'NONE',  ( 0.000000000000000000, 0.000000000000000000, 1.000000000000000000 ) ) ;
#75404=DIRECTION ( 'NONE',  ( 0.000000000000000000, 0.000000000000000000, 1.000000000000000000 ) ) ;
#75405=AXIS2_PLACEMENT_3D ( 'NONE', #60922, #11169, #41305 ) ;
#75406=DIRECTION ( 'NONE',  ( 0.000000000000000000, 1.000000000000000000, 0.000000000000000000 ) ) ;
#75407=EDGE_LOOP ( 'NONE', ( #103958, #78950, #92111, #70645 ) ) ;
#75408=AXIS2_PLACEMENT_3D ( 'NONE', #5391, #66242, #86530 ) ;
#75409=CIRCLE ( 'NONE', #8496, 0.09999999999999982514 ) ;
#75410=EDGE_CURVE ( 'NONE', #108949, #7522, #18480, .T. ) ;
#75411=CARTESIAN_POINT ( 'NONE',  ( -3.300000000000027800, 2.500000000000000000, -4.330127018922201643 ) ) ;
#75413=CARTESIAN_POINT ( 'NONE',  ( -5.650000000000019895, 12.50000000000000000, 6.841600689897072485 ) ) ;
#75415=ORIENTED_EDGE ( 'NONE', *, *, #124740, .F. ) ;
#75416=DIRECTION ( 'NONE',  ( 0.000000000000000000, 0.000000000000000000, -1.000000000000000000 ) ) ;
#75417=ORIENTED_EDGE ( 'NONE', *, *, #42005, .F. ) ;
#75418=CONICAL_SURFACE ( 'NONE', #6430, 0.09999999999999982514, 0.003490658503988666988 ) ;
#75419=VERTEX_POINT ( 'NONE', #38598 ) ;
#75420=LINE ( 'NONE', #55155, #84592 ) ;
#75421=DIRECTION ( 'NONE',  ( -0.000000000000000000, -1.000000000000000000, -0.000000000000000000 ) ) ;
#75422=CARTESIAN_POINT ( 'NONE',  ( -1.700000000000034817, 2.500000000000000000, -0.1000000000000023925 ) ) ;
#75423=CARTESIAN_POINT ( 'NONE',  ( -8.350000000000012079, 2.500000000000000000, 1.372243186433545370 ) ) ;
#75424=LINE ( 'NONE', #61931, #28238 ) ;
#75425=EDGE_LOOP ( 'NONE', ( #20020, #33393, #125308, #35469 ) ) ;
#75426=CARTESIAN_POINT ( 'NONE',  ( 0.1999999999999627909, 2.500000000000000000, 0.3464101615137758494 ) ) ;
#75427=DIRECTION ( 'NONE',  ( 0.000000000000000000, 1.000000000000000000, 0.000000000000000000 ) ) ;
#75428=ADVANCED_FACE ( 'NONE', ( #7813 ), #26898, .T. ) ;
#75429=LINE ( 'NONE', #76090, #89913 ) ;
#75430=DIRECTION ( 'NONE',  ( -0.000000000000000000, 1.000000000000000000, -0.000000000000000000 ) ) ;
#75431=CARTESIAN_POINT ( 'NONE',  ( 10.64999999999991331, 12.50000000000000000, -1.883746621131363375 ) ) ;
#75432=ORIENTED_EDGE ( 'NONE', *, *, #4771, .F. ) ;
#75433=CIRCLE ( 'NONE', #209, 0.06509327318403745899 ) ;
#75434=ORIENTED_EDGE ( 'NONE', *, *, #44102, .T. ) ;
#75435=EDGE_CURVE ( 'NONE', #40951, #108184, #49059, .T. ) ;
#75437=EDGE_CURVE ( 'NONE', #13624, #114894, #22710, .T. ) ;
#75438=ORIENTED_EDGE ( 'NONE', *, *, #121826, .F. ) ;
#75439=FACE_OUTER_BOUND ( 'NONE', #121247, .T. ) ;
#75440=AXIS2_PLACEMENT_3D ( 'NONE', #129564, #39882, #81087 ) ;
#75441=DIRECTION ( 'NONE',  ( 0.000000000000000000, 0.000000000000000000, -1.000000000000000000 ) ) ;
#75442=AXIS2_PLACEMENT_3D ( 'NONE', #79601, #110345, #118233 ) ;
#75443=EDGE_CURVE ( 'NONE', #96072, #65503, #78526, .T. ) ;
#75445=CARTESIAN_POINT ( 'NONE',  ( -11.44999999999999751, 2.500000000000000000, -2.511473670974873951 ) ) ;
#75446=CARTESIAN_POINT ( 'NONE',  ( -1.650000000000034328, 2.500000000000000000, -7.188010851410854052 ) ) ;
#75447=ADVANCED_FACE ( 'NONE', ( #128919 ), #12314, .T. ) ;
#75448=CARTESIAN_POINT ( 'NONE',  ( -3.550000000000031797, 2.500000000000000000, -6.148780366869526226 ) ) ;
#75449=FACE_OUTER_BOUND ( 'NONE', #15533, .T. ) ;
#75450=EDGE_LOOP ( 'NONE', ( #86298, #72294 ) ) ;
#75451=CIRCLE ( 'NONE', #50412, 0.1000000000000000472 ) ;
#75452=EDGE_CURVE ( 'NONE', #114600, #98683, #116856, .T. ) ;
#75453=CIRCLE ( 'NONE', #81712, 0.1000000000000002554 ) ;
#75454=EDGE_CURVE ( 'NONE', #70834, #54150, #50000, .T. ) ;
#75455=ADVANCED_FACE ( 'NONE', ( #117111 ), #85474, .T. ) ;
#75456=CARTESIAN_POINT ( 'NONE',  ( -10.45000000000000462, 2.500000000000000000, -2.265063509461097802 ) ) ;
#75457=LINE ( 'NONE', #63720, #76913 ) ;
#75458=ORIENTED_EDGE ( 'NONE', *, *, #99808, .T. ) ;
#75459=CARTESIAN_POINT ( 'NONE',  ( 11.44999999999990692, 2.500000000000000000, -6.941600689897078347 ) ) ;
#75460=DIRECTION ( 'NONE',  ( 0.000000000000000000, 0.000000000000000000, 1.000000000000000000 ) ) ;
#75461=EDGE_CURVE ( 'NONE', #60587, #85684, #99446, .T. ) ;
#75462=CARTESIAN_POINT ( 'NONE',  ( -8.750000000000010658, 2.500000000000000000, -1.572243186433550211 ) ) ;
#75463=CIRCLE ( 'NONE', #50342, 0.1000000000000002554 ) ;
#75464=AXIS2_PLACEMENT_3D ( 'NONE', #60691, #51509, #92056 ) ;
#75465=ORIENTED_EDGE ( 'NONE', *, *, #96847, .F. ) ;
#75467=PLANE ( 'NONE',  #88667 ) ;
#75468=ORIENTED_EDGE ( 'NONE', *, *, #17938, .T. ) ;
#75469=CARTESIAN_POINT ( 'NONE',  ( 6.049999999999932321, 2.500000000000000000, 6.741600689897071952 ) ) ;
#75470=DIRECTION ( 'NONE',  ( 0.000000000000000000, 0.000000000000000000, 1.000000000000000000 ) ) ;
#75471=AXIS2_PLACEMENT_3D ( 'NONE', #36390, #16701, #96558 ) ;
#75472=ORIENTED_EDGE ( 'NONE', *, *, #79610, .T. ) ;
#75473=DIRECTION ( 'NONE',  ( -0.000000000000000000, 1.000000000000000000, -0.000000000000000000 ) ) ;
#75474=CARTESIAN_POINT ( 'NONE',  ( 12.04999999999990479, 12.50000000000000000, -6.430097255199264339 ) ) ;
#75475=AXIS2_PLACEMENT_3D ( 'NONE', #98505, #67772, #90637 ) ;
#75477=ORIENTED_EDGE ( 'NONE', *, *, #20914, .T. ) ;
#75478=DIRECTION ( 'NONE',  ( 0.000000000000000000, 0.000000000000000000, 1.000000000000000000 ) ) ;
#75479=ORIENTED_EDGE ( 'NONE', *, *, #85992, .F. ) ;
#75480=ORIENTED_EDGE ( 'NONE', *, *, #59895, .F. ) ;
#75481=DIRECTION ( 'NONE',  ( -0.000000000000000000, -1.000000000000000000, -0.000000000000000000 ) ) ;
#75482=DIRECTION ( 'NONE',  ( 0.000000000000000000, 0.000000000000000000, -1.000000000000000000 ) ) ;
#75483=VERTEX_POINT ( 'NONE', #28768 ) ;
#75484=DIRECTION ( 'NONE',  ( 0.000000000000000000, 1.000000000000000000, 0.000000000000000000 ) ) ;
#75485=DIRECTION ( 'NONE',  ( -4.274815082592931898E-19, -0.9999939076577903929, -0.003490651415223739937 ) ) ;
#75486=ORIENTED_EDGE ( 'NONE', *, *, #64171, .T. ) ;
#75487=PLANE ( 'NONE',  #126149 ) ;
#75489=EDGE_CURVE ( 'NONE', #125527, #2669, #118925, .T. ) ;
#75490=AXIS2_PLACEMENT_3D ( 'NONE', #26162, #7140, #7796 ) ;
#75491=DIRECTION ( 'NONE',  ( 0.000000000000000000, 0.000000000000000000, 1.000000000000000000 ) ) ;
#75492=CARTESIAN_POINT ( 'NONE',  ( 13.09999999999990195, 12.50000000000000000, -3.983716857408426293 ) ) ;
#75493=AXIS2_PLACEMENT_3D ( 'NONE', #19058, #116631, #49213 ) ;
#75494=CARTESIAN_POINT ( 'NONE',  ( -15.19999999999998330, 2.500000000000000000, 0.4464101615137758272 ) ) ;
#75495=CARTESIAN_POINT ( 'NONE',  ( 0.1999999999999636513, 2.500000000000000000, -0.2464101615137760659 ) ) ;
#75496=CIRCLE ( 'NONE', #10731, 0.06509327318403745899 ) ;
#75497=ORIENTED_EDGE ( 'NONE', *, *, #109585, .F. ) ;
#75498=CIRCLE ( 'NONE', #60935, 0.06509327318403745899 ) ;
#75499=VERTEX_POINT ( 'NONE', #89610 ) ;
#75500=VERTEX_POINT ( 'NONE', #28114 ) ;
#75501=EDGE_LOOP ( 'NONE', ( #1202, #33162 ) ) ;
#75502=FACE_OUTER_BOUND ( 'NONE', #93104, .T. ) ;
#75503=CARTESIAN_POINT ( 'NONE',  ( 8.549999999999924327, 2.500000000000000000, 1.818653347947321475 ) ) ;
#75504=AXIS2_PLACEMENT_3D ( 'NONE', #76858, #116764, #57866 ) ;
#75505=CARTESIAN_POINT ( 'NONE',  ( 11.24999999999990941, 2.500000000000000000, 7.188010851410848723 ) ) ;
#75506=ORIENTED_EDGE ( 'NONE', *, *, #113831, .T. ) ;
#75507=EDGE_CURVE ( 'NONE', #7967, #99945, #68029, .T. ) ;
#75508=FACE_BOUND ( 'NONE', #81506, .T. ) ;
#75509=FACE_OUTER_BOUND ( 'NONE', #19556, .T. ) ;
#75510=DIRECTION ( 'NONE',  ( 0.000000000000000000, 0.000000000000000000, 1.000000000000000000 ) ) ;
#75511=FACE_OUTER_BOUND ( 'NONE', #49750, .T. ) ;
#75512=FACE_OUTER_BOUND ( 'NONE', #62283, .T. ) ;
#75513=PLANE ( 'NONE',  #95288 ) ;
#75514=DIRECTION ( 'NONE',  ( 0.000000000000000000, -0.9999939076577903929, 0.003490651415223739937 ) ) ;
#75515=DIRECTION ( 'NONE',  ( 0.000000000000000000, 0.000000000000000000, 1.000000000000000000 ) ) ;
#75516=DIRECTION ( 'NONE',  ( 0.000000000000000000, 1.000000000000000000, 0.000000000000000000 ) ) ;
#75517=DIRECTION ( 'NONE',  ( 0.000000000000000000, 0.000000000000000000, 1.000000000000000000 ) ) ;
#75518=CARTESIAN_POINT ( 'NONE',  ( -5.400000000000019895, 2.500000000000000000, 4.330127018922196314 ) ) ;
#75519=ORIENTED_EDGE ( 'NONE', *, *, #13009, .T. ) ;
#75520=ORIENTED_EDGE ( 'NONE', *, *, #86630, .F. ) ;
#75521=VERTEX_POINT ( 'NONE', #18281 ) ;
#75522=ORIENTED_EDGE ( 'NONE', *, *, #124031, .T. ) ;
#75523=DIRECTION ( 'NONE',  ( 0.000000000000000000, 0.000000000000000000, 1.000000000000000000 ) ) ;
#75524=EDGE_LOOP ( 'NONE', ( #91811, #67079 ) ) ;
#75525=DIRECTION ( 'NONE',  ( 0.000000000000000000, 1.000000000000000000, 0.000000000000000000 ) ) ;
#75526=VERTEX_POINT ( 'NONE', #40534 ) ;
#75527=ORIENTED_EDGE ( 'NONE', *, *, #55192, .T. ) ;
#75528=CARTESIAN_POINT ( 'NONE',  ( -3.100000000000028511, 12.50000000000000000, -3.983716857408426293 ) ) ;
#75529=CONICAL_SURFACE ( 'NONE', #40046, 0.1000000000000002554, 0.003490658503988666988 ) ;
#75530=AXIS2_PLACEMENT_3D ( 'NONE', #59176, #70919, #110826 ) ;
#75531=EDGE_CURVE ( 'NONE', #47341, #100839, #52041, .T. ) ;
#75532=CARTESIAN_POINT ( 'NONE',  ( 8.340322510127135658, -2.499999999999999556, 8.517653997967773449 ) ) ;
#75533=LINE ( 'NONE', #65723, #93833 ) ;
#75534=CARTESIAN_POINT ( 'NONE',  ( 13.94999999999989626, 2.500000000000000000, 2.611473670974873151 ) ) ;
#75535=CARTESIAN_POINT ( 'NONE',  ( 6.649999999999927525, 2.500000000000000000, 2.165063509461097713 ) ) ;
#75536=EDGE_LOOP ( 'NONE', ( #50327, #27128, #84036, #92239 ) ) ;
#75537=CONICAL_SURFACE ( 'NONE', #100669, 0.09999999999999999167, 0.003490658503988666988 ) ;
#75538=ADVANCED_FACE ( 'NONE', ( #81710 ), #113108, .T. ) ;
#75539=AXIS2_PLACEMENT_3D ( 'NONE', #34052, #111974, #25495 ) ;
#75540=ORIENTED_EDGE ( 'NONE', *, *, #78274, .T. ) ;
#75541=EDGE_LOOP ( 'NONE', ( #95900, #88406 ) ) ;
#75542=ORIENTED_EDGE ( 'NONE', *, *, #76780, .T. ) ;
#75543=ADVANCED_FACE ( 'NONE', ( #31994 ), #81387, .T. ) ;
#75545=EDGE_CURVE ( 'NONE', #11304, #4486, #106400, .T. ) ;
#75546=ADVANCED_FACE ( 'NONE', ( #111156 ), #110606, .T. ) ;
#75547=ORIENTED_EDGE ( 'NONE', *, *, #14288, .T. ) ;
#75548=EDGE_CURVE ( 'NONE', #118876, #91012, #22182, .T. ) ;
#75549=ORIENTED_EDGE ( 'NONE', *, *, #40718, .F. ) ;
#75550=CIRCLE ( 'NONE', #102737, 0.09999999999999999167 ) ;
#75551=CARTESIAN_POINT ( 'NONE',  ( -11.44999999999999751, 2.500000000000000000, 6.841600689897072485 ) ) ;
#75553=AXIS2_PLACEMENT_3D ( 'NONE', #21900, #1584, #109627 ) ;
#75554=CARTESIAN_POINT ( 'NONE',  ( -12.09999999999999609, 12.50000000000000000, -5.022947341949751454 ) ) ;
#75555=CARTESIAN_POINT ( 'NONE',  ( -12.49999999999995914, 2.500000000000000000, 0.1000000000000018513 ) ) ;
#75556=LINE ( 'NONE', #23905, #108854 ) ;
#75557=AXIS2_PLACEMENT_3D ( 'NONE', #26522, #54049, #25874 ) ;
#75558=PLANE ( 'NONE',  #56608 ) ;
#75559=CARTESIAN_POINT ( 'NONE',  ( 13.94999999999989626, 12.50000000000000000, 2.511473670974873507 ) ) ;
#75560=EDGE_CURVE ( 'NONE', #40528, #30572, #3987, .T. ) ;
#75561=VECTOR ( 'NONE', #47484, 1000.000000000000000 ) ;
#75562=VERTEX_POINT ( 'NONE', #122306 ) ;
#75563=CARTESIAN_POINT ( 'NONE',  ( -8.550000000000013145, 12.50000000000000000, -1.883746621131363597 ) ) ;
#75564=EDGE_CURVE ( 'NONE', #27825, #5027, #54188, .T. ) ;
#75566=VERTEX_POINT ( 'NONE', #80443 ) ;
#75567=FACE_OUTER_BOUND ( 'NONE', #25439, .T. ) ;
#75568=ORIENTED_EDGE ( 'NONE', *, *, #17766, .F. ) ;
#75569=CARTESIAN_POINT ( 'NONE',  ( -1.650000000000034772, 2.500000000000000000, 5.902370205355745192 ) ) ;
#75570=CIRCLE ( 'NONE', #44180, 10.00000000000000000 ) ;
#75571=LINE ( 'NONE', #46777, #13524 ) ;
#75572=EDGE_LOOP ( 'NONE', ( #32704, #108621, #62683, #21668 ) ) ;
#75573=CARTESIAN_POINT ( 'NONE',  ( -2.900000000000029665, 2.500000000000000000, 4.230127018922196669 ) ) ;
#75575=ORIENTED_EDGE ( 'NONE', *, *, #105553, .T. ) ;
#75576=DIRECTION ( 'NONE',  ( 0.000000000000000000, 1.000000000000000000, 0.000000000000000000 ) ) ;
#75577=PLANE ( 'NONE',  #19426 ) ;
#75578=EDGE_LOOP ( 'NONE', ( #32676, #30218, #80370, #34544 ) ) ;
#75579=ORIENTED_EDGE ( 'NONE', *, *, #15566, .F. ) ;
#75580=CARTESIAN_POINT ( 'NONE',  ( -0.4000000000000331624, 12.50000000000000000, -0.6277270498435144619 ) ) ;
#75581=FACE_OUTER_BOUND ( 'NONE', #4843, .T. ) ;
#75584=CARTESIAN_POINT ( 'NONE',  ( 9.399999999999915090, 12.50000000000000000, -4.741630453620015118 ) ) ;
#75585=DIRECTION ( 'NONE',  ( 0.000000000000000000, 1.000000000000000000, 0.000000000000000000 ) ) ;
#75586=CIRCLE ( 'NONE', #125749, 0.09999999999999982514 ) ;
#75587=AXIS2_PLACEMENT_3D ( 'NONE', #6631, #106171, #8582 ) ;
#75588=EDGE_LOOP ( 'NONE', ( #65837, #63221, #93914, #42662 ) ) ;
#75589=DIRECTION ( 'NONE',  ( -0.000000000000000000, 1.000000000000000000, -0.000000000000000000 ) ) ;
#75590=VECTOR ( 'NONE', #101802, 1000.000000000000000 ) ;
#75591=EDGE_LOOP ( 'NONE', ( #17733, #93130, #27631, #12288 ) ) ;
#75592=CIRCLE ( 'NONE', #117430, 0.1000000000000002554 ) ;
#75593=DIRECTION ( 'NONE',  ( 0.000000000000000000, 1.000000000000000000, 0.000000000000000000 ) ) ;
#75594=DIRECTION ( 'NONE',  ( 0.000000000000000000, 0.000000000000000000, 1.000000000000000000 ) ) ;
#75595=EDGE_CURVE ( 'NONE', #102282, #56299, #29064, .T. ) ;
#75596=FACE_OUTER_BOUND ( 'NONE', #100361, .T. ) ;
#75597=ORIENTED_EDGE ( 'NONE', *, *, #33937, .T. ) ;
#75598=CIRCLE ( 'NONE', #117438, 0.06509327318403745899 ) ;
#75599=EDGE_CURVE ( 'NONE', #126826, #71554, #93897, .T. ) ;
#75600=ADVANCED_FACE ( 'NONE', ( #53557 ), #45781, .T. ) ;
#75601=CARTESIAN_POINT ( 'NONE',  ( -14.79999999999998295, 2.500000000000000000, -0.4464101615137760493 ) ) ;
#75603=ORIENTED_EDGE ( 'NONE', *, *, #103490, .T. ) ;
#75604=ADVANCED_FACE ( 'NONE', ( #1225 ), #41681, .T. ) ;
#75605=DIRECTION ( 'NONE',  ( -0.000000000000000000, -1.000000000000000000, -0.000000000000000000 ) ) ;
#75606=ORIENTED_EDGE ( 'NONE', *, *, #3585, .F. ) ;
#75607=EDGE_LOOP ( 'NONE', ( #38177, #89822 ) ) ;
#75608=DIRECTION ( 'NONE',  ( 0.000000000000000000, 0.000000000000000000, -1.000000000000000000 ) ) ;
#75609=ORIENTED_EDGE ( 'NONE', *, *, #87692, .F. ) ;
#75610=CARTESIAN_POINT ( 'NONE',  ( -0.6500000000000389910, 12.50000000000000000, -6.213873640053564351 ) ) ;
#75611=CARTESIAN_POINT ( 'NONE',  ( -4.800000000000022915, 2.500000000000000000, -0.3464101615137783474 ) ) ;
#75612=FACE_OUTER_BOUND ( 'NONE', #95517, .T. ) ;
#75613=VECTOR ( 'NONE', #112958, 1000.000000000000000 ) ;
#75614=ORIENTED_EDGE ( 'NONE', *, *, #22360, .T. ) ;
#75616=FACE_BOUND ( 'NONE', #93380, .T. ) ;
#75617=DIRECTION ( 'NONE',  ( -4.274815082592931898E-19, -0.9999939076577903929, -0.003490651415223739937 ) ) ;
#75618=VERTEX_POINT ( 'NONE', #71248 ) ;
#75619=PLANE ( 'NONE',  #33977 ) ;
#75620=CARTESIAN_POINT ( 'NONE',  ( -10.20000000000000462, 2.500000000000000000, -4.776537180435973085 ) ) ;
#75621=EDGE_CURVE ( 'NONE', #61759, #20290, #6043, .T. ) ;
#75622=AXIS2_PLACEMENT_3D ( 'NONE', #118296, #129439, #58739 ) ;
#75623=ORIENTED_EDGE ( 'NONE', *, *, #125123, .T. ) ;
#75624=VECTOR ( 'NONE', #86535, 1000.000000000000000 ) ;
#75625=AXIS2_PLACEMENT_3D ( 'NONE', #64493, #4261, #44200 ) ;
#75626=EDGE_LOOP ( 'NONE', ( #121266, #22955 ) ) ;
#75627=AXIS2_PLACEMENT_3D ( 'NONE', #92435, #2765, #32897 ) ;
#75628=ORIENTED_EDGE ( 'NONE', *, *, #66593, .F. ) ;
#75629=CARTESIAN_POINT ( 'NONE',  ( -11.44999999999999751, 12.50000000000000000, 6.841600689897072485 ) ) ;
#75630=FACE_OUTER_BOUND ( 'NONE', #77542, .T. ) ;
#75631=LINE ( 'NONE', #54080, #39992 ) ;
#75632=FACE_BOUND ( 'NONE', #22719, .T. ) ;
#75633=ORIENTED_EDGE ( 'NONE', *, *, #9069, .F. ) ;
#75635=DIRECTION ( 'NONE',  ( 0.000000000000000000, -0.000000000000000000, 1.000000000000000000 ) ) ;
#75636=DIRECTION ( 'NONE',  ( -0.000000000000000000, -1.000000000000000000, -0.000000000000000000 ) ) ;
#75637=AXIS2_PLACEMENT_3D ( 'NONE', #83531, #73686, #113625 ) ;
#75638=CIRCLE ( 'NONE', #106944, 0.06509327318403745899 ) ;
#75639=LINE ( 'NONE', #35109, #105648 ) ;
#75640=ADVANCED_FACE ( 'NONE', ( #63376 ), #570, .T. ) ;
#75641=VECTOR ( 'NONE', #126542, 1000.000000000000000 ) ;
#75642=CIRCLE ( 'NONE', #19208, 0.1000000000000002554 ) ;
#75643=AXIS2_PLACEMENT_3D ( 'NONE', #25280, #14175, #25954 ) ;
#75644=DIRECTION ( 'NONE',  ( -0.000000000000000000, -1.000000000000000000, -0.000000000000000000 ) ) ;
#75645=DIRECTION ( 'NONE',  ( -4.274815082592931898E-19, -0.9999939076577903929, -0.003490651415223739937 ) ) ;
#75646=DIRECTION ( 'NONE',  ( 0.000000000000000000, 1.000000000000000000, 0.000000000000000000 ) ) ;
#75647=CONICAL_SURFACE ( 'NONE', #107042, 0.09999999999999982514, 0.003490658503988666988 ) ;
#75648=FACE_OUTER_BOUND ( 'NONE', #84639, .T. ) ;
#75649=DIRECTION ( 'NONE',  ( 0.000000000000000000, 0.000000000000000000, 1.000000000000000000 ) ) ;
#75650=ORIENTED_EDGE ( 'NONE', *, *, #28461, .F. ) ;
#75651=AXIS2_PLACEMENT_3D ( 'NONE', #50546, #90465, #32875 ) ;
#75652=ORIENTED_EDGE ( 'NONE', *, *, #125934, .T. ) ;
#75653=ORIENTED_EDGE ( 'NONE', *, *, #63015, .F. ) ;
#75655=ORIENTED_EDGE ( 'NONE', *, *, #4619, .F. ) ;
#75656=CARTESIAN_POINT ( 'NONE',  ( 14.14999999999989377, 2.500000000000000000, -2.857883832488653741 ) ) ;
#75657=DIRECTION ( 'NONE',  ( 0.000000000000000000, -0.000000000000000000, 1.000000000000000000 ) ) ;
#75658=ORIENTED_EDGE ( 'NONE', *, *, #95206, .T. ) ;
#75659=EDGE_CURVE ( 'NONE', #102047, #1314, #121078, .T. ) ;
#75660=FACE_BOUND ( 'NONE', #124575, .T. ) ;
#75661=DIRECTION ( 'NONE',  ( -0.000000000000000000, -1.000000000000000000, -0.000000000000000000 ) ) ;
#75663=DIRECTION ( 'NONE',  ( 1.000000000000000000, 0.000000000000000000, 0.000000000000000000 ) ) ;
#75664=EDGE_CURVE ( 'NONE', #127955, #65687, #43742, .T. ) ;
#75665=FACE_OUTER_BOUND ( 'NONE', #30163, .T. ) ;
#75666=DIRECTION ( 'NONE',  ( 0.000000000000000000, 0.000000000000000000, 1.000000000000000000 ) ) ;
#75667=ORIENTED_EDGE ( 'NONE', *, *, #71100, .T. ) ;
#75669=VERTEX_POINT ( 'NONE', #87981 ) ;
#75670=ORIENTED_EDGE ( 'NONE', *, *, #97021, .T. ) ;
#75671=AXIS2_PLACEMENT_3D ( 'NONE', #113652, #63910, #78256 ) ;
#75672=EDGE_LOOP ( 'NONE', ( #75048, #19825, #68077, #89677 ) ) ;
#75673=AXIS2_PLACEMENT_3D ( 'NONE', #19683, #20965, #99541 ) ;
#75674=CARTESIAN_POINT ( 'NONE',  ( 13.94999999999989271, 12.50000000000000000, -1.818653347947326138 ) ) ;
#75675=CARTESIAN_POINT ( 'NONE',  ( -12.69999999999999041, 2.500000000000000000, 3.883716857408421319 ) ) ;
#75676=DIRECTION ( 'NONE',  ( 0.000000000000000000, 1.000000000000000000, 0.000000000000000000 ) ) ;
#75677=ORIENTED_EDGE ( 'NONE', *, *, #99580, .T. ) ;
#75678=CARTESIAN_POINT ( 'NONE',  ( 3.710216157338618537, 1.500000000000638156, -9.999999999999998224 ) ) ;
#75679=DIRECTION ( 'NONE',  ( -4.274815082592931898E-19, -0.9999939076577903929, -0.003490651415223739937 ) ) ;
#75680=CIRCLE ( 'NONE', #100724, 0.09999999999999982514 ) ;
#75681=CIRCLE ( 'NONE', #119600, 0.06509327318403745899 ) ;
#75682=CIRCLE ( 'NONE', #121754, 0.1000000000000002554 ) ;
#75683=EDGE_CURVE ( 'NONE', #124666, #102847, #114395, .T. ) ;
#75684=DIRECTION ( 'NONE',  ( 0.000000000000000000, 0.000000000000000000, -1.000000000000000000 ) ) ;
#75687=CONICAL_SURFACE ( 'NONE', #19247, 0.1000000000000000056, 0.003490658503988666988 ) ;
#75688=CIRCLE ( 'NONE', #19248, 0.06509327318403745899 ) ;
#75689=CARTESIAN_POINT ( 'NONE',  ( 3.099999999999944134, 2.500000000000000000, 4.576537180435972019 ) ) ;
#75690=ORIENTED_EDGE ( 'NONE', *, *, #122553, .T. ) ;
#75691=DIRECTION ( 'NONE',  ( 0.000000000000000000, 1.000000000000000000, 0.000000000000000000 ) ) ;
#75692=CONICAL_SURFACE ( 'NONE', #19255, 0.09999999999999999167, 0.003490658503988666988 ) ;
#75693=EDGE_CURVE ( 'NONE', #60634, #95189, #112672, .T. ) ;
#75694=VERTEX_POINT ( 'NONE', #35218 ) ;
#75695=EDGE_LOOP ( 'NONE', ( #10841, #114587 ) ) ;
#75697=EDGE_CURVE ( 'NONE', #129522, #1501, #83663, .T. ) ;
#75698=LINE ( 'NONE', #63964, #17424 ) ;
#75699=DIRECTION ( 'NONE',  ( 0.000000000000000000, -0.000000000000000000, 1.000000000000000000 ) ) ;
#75700=EDGE_CURVE ( 'NONE', #110514, #21869, #70912, .T. ) ;
#75701=EDGE_CURVE ( 'NONE', #35149, #11533, #67708, .T. ) ;
#75702=EDGE_CURVE ( 'NONE', #105674, #14788, #4415, .T. ) ;
#75703=ORIENTED_EDGE ( 'NONE', *, *, #78097, .T. ) ;
#75704=EDGE_LOOP ( 'NONE', ( #53189, #54373 ) ) ;
#75705=CARTESIAN_POINT ( 'NONE',  ( 3.749999999999942268, 12.50000000000000000, 1.472243186433545459 ) ) ;
#75706=CARTESIAN_POINT ( 'NONE',  ( 3.149999999999944400, 2.500000000000000000, 2.611473670974873151 ) ) ;
#75707=EDGE_CURVE ( 'NONE', #84904, #6379, #35317, .T. ) ;
#75708=DIRECTION ( 'NONE',  ( 0.000000000000000000, 0.000000000000000000, 1.000000000000000000 ) ) ;
#75709=VERTEX_POINT ( 'NONE', #33912 ) ;
#75710=EDGE_LOOP ( 'NONE', ( #101896, #76138 ) ) ;
#75711=ADVANCED_FACE ( 'NONE', ( #24737 ), #57914, .T. ) ;
#75712=DIRECTION ( 'NONE',  ( 0.000000000000000000, 0.000000000000000000, -1.000000000000000000 ) ) ;
#75713=ADVANCED_FACE ( 'NONE', ( #84939 ), #73833, .T. ) ;
#75714=AXIS2_PLACEMENT_3D ( 'NONE', #76419, #56113, #116318 ) ;
#75715=ORIENTED_EDGE ( 'NONE', *, *, #13020, .T. ) ;
#75716=DIRECTION ( 'NONE',  ( 0.000000000000000000, 1.000000000000000000, 0.000000000000000000 ) ) ;
#75717=ADVANCED_FACE ( 'NONE', ( #37630 ), #108451, .T. ) ;
#75718=ADVANCED_FACE ( 'NONE', ( #17295 ), #57261, .T. ) ;
#75719=FACE_OUTER_BOUND ( 'NONE', #74105, .T. ) ;
#75720=ORIENTED_EDGE ( 'NONE', *, *, #2644, .T. ) ;
#75721=DIRECTION ( 'NONE',  ( 0.000000000000000000, -0.000000000000000000, 1.000000000000000000 ) ) ;
#75722=FACE_OUTER_BOUND ( 'NONE', #105290, .T. ) ;
#75723=DIRECTION ( 'NONE',  ( 0.000000000000000000, 1.000000000000000000, 0.000000000000000000 ) ) ;
#75724=DIRECTION ( 'NONE',  ( 0.000000000000000000, 0.000000000000000000, -1.000000000000000000 ) ) ;
#75725=AXIS2_PLACEMENT_3D ( 'NONE', #43621, #25232, #106383 ) ;
#75726=EDGE_CURVE ( 'NONE', #18013, #109495, #113769, .T. ) ;
#75727=ORIENTED_EDGE ( 'NONE', *, *, #110973, .F. ) ;
#75728=CARTESIAN_POINT ( 'NONE',  ( 3.749999999999942268, 2.500000000000000000, -1.472243186433550122 ) ) ;
#75729=AXIS2_PLACEMENT_3D ( 'NONE', #79486, #90574, #119383 ) ;
#75730=CARTESIAN_POINT ( 'NONE',  ( 6.849999999999927702, 2.500000000000000000, 1.718653347947321386 ) ) ;
#75731=VERTEX_POINT ( 'NONE', #103943 ) ;
#75732=ORIENTED_EDGE ( 'NONE', *, *, #87527, .T. ) ;
#75734=CARTESIAN_POINT ( 'NONE',  ( 12.69999999999990337, 12.50000000000000000, -4.611443907251940644 ) ) ;
#75735=LINE ( 'NONE', #115658, #30134 ) ;
#75736=CARTESIAN_POINT ( 'NONE',  ( -6.050000000000017586, 2.500000000000000000, 6.148780366869520009 ) ) ;
#75738=LINE ( 'NONE', #85566, #115843 ) ;
#75739=DIRECTION ( 'NONE',  ( 0.000000000000000000, -0.9999939076577903929, 0.003490651415223739937 ) ) ;
#75740=AXIS2_PLACEMENT_3D ( 'NONE', #11252, #9327, #100298 ) ;
#75741=FACE_OUTER_BOUND ( 'NONE', #46557, .T. ) ;
#75742=AXIS2_PLACEMENT_3D ( 'NONE', #105995, #16926, #86992 ) ;
#75743=DIRECTION ( 'NONE',  ( 0.000000000000000000, 1.000000000000000000, 0.000000000000000000 ) ) ;
#75744=CONICAL_SURFACE ( 'NONE', #79954, 0.09999999999999982514, 0.003490658503988666988 ) ;
#75745=CIRCLE ( 'NONE', #123757, 0.1000000000000002554 ) ;
#75746=LINE ( 'NONE', #16162, #19137 ) ;
#75747=AXIS2_PLACEMENT_3D ( 'NONE', #109962, #108656, #18979 ) ;
#75748=DIRECTION ( 'NONE',  ( 0.000000000000000000, 0.000000000000000000, 1.000000000000000000 ) ) ;
#75749=ORIENTED_EDGE ( 'NONE', *, *, #80935, .F. ) ;
#75750=AXIS2_PLACEMENT_3D ( 'NONE', #55566, #75833, #5157 ) ;
#75751=ORIENTED_EDGE ( 'NONE', *, *, #119486, .F. ) ;
#75752=ORIENTED_EDGE ( 'NONE', *, *, #21842, .T. ) ;
#75753=CARTESIAN_POINT ( 'NONE',  ( 9.599999999999914380, 2.500000000000000000, -3.737306695894649700 ) ) ;
#75754=FACE_OUTER_BOUND ( 'NONE', #45386, .T. ) ;
#75755=DIRECTION ( 'NONE',  ( 0.000000000000000000, 1.000000000000000000, 0.000000000000000000 ) ) ;
#75756=ORIENTED_EDGE ( 'NONE', *, *, #53473, .F. ) ;
#75757=DIRECTION ( 'NONE',  ( 0.000000000000000000, 0.000000000000000000, -1.000000000000000000 ) ) ;
#75758=EDGE_CURVE ( 'NONE', #34246, #28179, #34578, .T. ) ;
#75759=EDGE_CURVE ( 'NONE', #72461, #72089, #7500, .T. ) ;
#75760=CARTESIAN_POINT ( 'NONE',  ( 4.199999999999938005, 12.50000000000000000, 4.330127018922196314 ) ) ;
#75761=DIRECTION ( 'NONE',  ( -0.000000000000000000, 1.000000000000000000, -0.000000000000000000 ) ) ;
#75762=EDGE_LOOP ( 'NONE', ( #99187, #118734, #108723, #23738 ) ) ;
#75763=CIRCLE ( 'NONE', #105307, 0.06509327318403745899 ) ;
#75764=CARTESIAN_POINT ( 'NONE',  ( 9.599999999999914380, 2.500000000000000000, -3.637306695894650055 ) ) ;
#75765=VERTEX_POINT ( 'NONE', #87339 ) ;
#75766=EDGE_CURVE ( 'NONE', #123488, #102877, #77530, .T. ) ;
#75767=ORIENTED_EDGE ( 'NONE', *, *, #19811, .T. ) ;
#75768=VERTEX_POINT ( 'NONE', #28452 ) ;
#75769=AXIS2_PLACEMENT_3D ( 'NONE', #63103, #123314, #43484 ) ;
#75770=ORIENTED_EDGE ( 'NONE', *, *, #46470, .T. ) ;
#75771=DIRECTION ( 'NONE',  ( 0.000000000000000000, 1.000000000000000000, 0.000000000000000000 ) ) ;
#75772=AXIS2_PLACEMENT_3D ( 'NONE', #47745, #37285, #126947 ) ;
#75773=DIRECTION ( 'NONE',  ( -4.274815082592931898E-19, -0.9999939076577903929, -0.003490651415223739937 ) ) ;
#75774=CARTESIAN_POINT ( 'NONE',  ( 1.049999999999952083, 12.50000000000000000, 6.776507416713035248 ) ) ;
#75775=DIRECTION ( 'NONE',  ( 0.000000000000000000, -0.9999939076577903929, 0.003490651415223739937 ) ) ;
#75776=CIRCLE ( 'NONE', #67431, 0.1000000000000000472 ) ;
#75777=ORIENTED_EDGE ( 'NONE', *, *, #93483, .T. ) ;
#75778=AXIS2_PLACEMENT_3D ( 'NONE', #119076, #1228, #28116 ) ;
#75779=CIRCLE ( 'NONE', #69429, 0.1000000000000002554 ) ;
#75780=CARTESIAN_POINT ( 'NONE',  ( -9.400000000000007461, 12.50000000000000000, 3.918623584224382839 ) ) ;
#75781=AXIS2_PLACEMENT_3D ( 'NONE', #119983, #41442, #110162 ) ;
#75782=ORIENTED_EDGE ( 'NONE', *, *, #23540, .T. ) ;
#75783=CARTESIAN_POINT ( 'NONE',  ( 6.649999999999929301, 2.500000000000000000, -2.065063509461102065 ) ) ;
#75784=DIRECTION ( 'NONE',  ( 0.000000000000000000, 1.000000000000000000, 0.000000000000000000 ) ) ;
#75785=CARTESIAN_POINT ( 'NONE',  ( -2.500000000000031086, 2.500000000000000000, 3.637306695894644726 ) ) ;
#75786=DIRECTION ( 'NONE',  ( 0.000000000000000000, 1.000000000000000000, 0.000000000000000000 ) ) ;
#75787=CIRCLE ( 'NONE', #46539, 0.1000000000000002554 ) ;
#75788=ORIENTED_EDGE ( 'NONE', *, *, #117055, .T. ) ;
#75789=VERTEX_POINT ( 'NONE', #108283 ) ;
#75790=VERTEX_POINT ( 'NONE', #68356 ) ;
#75791=DIRECTION ( 'NONE',  ( 0.000000000000000000, 1.000000000000000000, 0.000000000000000000 ) ) ;
#75792=CARTESIAN_POINT ( 'NONE',  ( 3.749999999999940492, 2.500000000000000000, 5.802370205355744659 ) ) ;
#75793=CARTESIAN_POINT ( 'NONE',  ( 0.3999999999999568345, 12.50000000000000000, -3.572213422710612374 ) ) ;
#75794=FACE_BOUND ( 'NONE', #998, .T. ) ;
#75795=DIRECTION ( 'NONE',  ( -0.000000000000000000, 1.000000000000000000, -0.000000000000000000 ) ) ;
#75796=DIRECTION ( 'NONE',  ( 0.000000000000000000, 0.000000000000000000, -1.000000000000000000 ) ) ;
#75797=CARTESIAN_POINT ( 'NONE',  ( 13.54999999999989768, 2.500000000000000000, -2.511473670974877948 ) ) ;
#75798=FACE_OUTER_BOUND ( 'NONE', #38599, .T. ) ;
#75799=AXIS2_PLACEMENT_3D ( 'NONE', #59238, #99149, #89320 ) ;
#75800=ADVANCED_FACE ( 'NONE', ( #18616 ), #116946, .T. ) ;
#75802=DIRECTION ( 'NONE',  ( 0.000000000000000000, 0.000000000000000000, -1.000000000000000000 ) ) ;
#75803=CARTESIAN_POINT ( 'NONE',  ( -7.500000000000016875, 12.50000000000000000, -3.572213422710612374 ) ) ;
#75804=AXIS2_PLACEMENT_3D ( 'NONE', #27154, #36981, #86721 ) ;
#75806=CIRCLE ( 'NONE', #29856, 0.1000000000000002554 ) ;
#75807=DIRECTION ( 'NONE',  ( 0.000000000000000000, 0.000000000000000000, 1.000000000000000000 ) ) ;
#75808=ORIENTED_EDGE ( 'NONE', *, *, #35738, .F. ) ;
#75809=ORIENTED_EDGE ( 'NONE', *, *, #7098, .T. ) ;
#75810=ORIENTED_EDGE ( 'NONE', *, *, #60978, .F. ) ;
#75811=ORIENTED_EDGE ( 'NONE', *, *, #32112, .T. ) ;
#75812=EDGE_CURVE ( 'NONE', #34635, #71492, #6135, .T. ) ;
#75814=EDGE_CURVE ( 'NONE', #13385, #49583, #102308, .T. ) ;
#75815=FACE_BOUND ( 'NONE', #4098, .T. ) ;
#75816=AXIS2_PLACEMENT_3D ( 'NONE', #127015, #45877, #37348 ) ;
#75817=CARTESIAN_POINT ( 'NONE',  ( -3.550000000000027356, 12.50000000000000000, -2.511473670974877948 ) ) ;
#75818=CIRCLE ( 'NONE', #38279, 0.1000000000000002554 ) ;
#75819=AXIS2_PLACEMENT_3D ( 'NONE', #21774, #41426, #109500 ) ;
#75820=AXIS2_PLACEMENT_3D ( 'NONE', #9450, #49390, #110225 ) ;
#75821=EDGE_LOOP ( 'NONE', ( #80437, #5165 ) ) ;
#75822=CARTESIAN_POINT ( 'NONE',  ( 32.28071041560450993, 1.401423001988622019, 4.680142630335600629 ) ) ;
#75823=ADVANCED_FACE ( 'NONE', ( #70942 ), #41771, .T. ) ;
#75824=DIRECTION ( 'NONE',  ( -0.000000000000000000, -1.000000000000000000, -0.000000000000000000 ) ) ;
#75826=AXIS2_PLACEMENT_3D ( 'NONE', #10441, #88334, #120408 ) ;
#75827=LINE ( 'NONE', #115755, #55331 ) ;
#75828=DIRECTION ( 'NONE',  ( -0.000000000000000000, -1.000000000000000000, -0.000000000000000000 ) ) ;
#75829=VECTOR ( 'NONE', #41789, 1000.000000000000000 ) ;
#75830=CONICAL_SURFACE ( 'NONE', #128174, 0.09999999999999999167, 0.003490658503988666988 ) ;
#75831=CIRCLE ( 'NONE', #4717, 0.06509327318403745899 ) ;
#75832=EDGE_LOOP ( 'NONE', ( #101869, #40886 ) ) ;
#75833=DIRECTION ( 'NONE',  ( -0.000000000000000000, -1.000000000000000000, -0.000000000000000000 ) ) ;
#75834=DIRECTION ( 'NONE',  ( 0.000000000000000000, 0.000000000000000000, 1.000000000000000000 ) ) ;
#75835=ORIENTED_EDGE ( 'NONE', *, *, #28176, .T. ) ;
#75836=DIRECTION ( 'NONE',  ( 0.000000000000000000, 0.000000000000000000, 1.000000000000000000 ) ) ;
#75837=AXIS2_PLACEMENT_3D ( 'NONE', #117030, #48983, #27367 ) ;
#75838=DIRECTION ( 'NONE',  ( 0.000000000000000000, 0.000000000000000000, 1.000000000000000000 ) ) ;
#75839=VERTEX_POINT ( 'NONE', #10089 ) ;
#75840=FACE_OUTER_BOUND ( 'NONE', #30732, .T. ) ;
#75842=ORIENTED_EDGE ( 'NONE', *, *, #35672, .T. ) ;
#75843=FACE_OUTER_BOUND ( 'NONE', #22599, .T. ) ;
#75844=VERTEX_POINT ( 'NONE', #50656 ) ;
#75845=CARTESIAN_POINT ( 'NONE',  ( -13.34999999999999076, 2.500000000000000000, -1.472243186433547901 ) ) ;
#75846=DIRECTION ( 'NONE',  ( 0.000000000000000000, 0.000000000000000000, 1.000000000000000000 ) ) ;
#75847=EDGE_CURVE ( 'NONE', #127429, #3902, #4086, .T. ) ;
#75848=VERTEX_POINT ( 'NONE', #253 ) ;
#75849=DIRECTION ( 'NONE',  ( -0.000000000000000000, 1.000000000000000000, -0.000000000000000000 ) ) ;
#75851=DIRECTION ( 'NONE',  ( 0.000000000000000000, 1.000000000000000000, 0.000000000000000000 ) ) ;
#75852=CIRCLE ( 'NONE', #115855, 0.09999999999999982514 ) ;
#75853=DIRECTION ( 'NONE',  ( -4.274815082592931898E-19, -0.9999939076577903929, -0.003490651415223739937 ) ) ;
#75854=CONICAL_SURFACE ( 'NONE', #115551, 0.1000000000000002554, 0.003490658503988666988 ) ;
#75855=CARTESIAN_POINT ( 'NONE',  ( -11.44999999999999929, 2.500000000000000000, -6.148780366869522673 ) ) ;
#75856=EDGE_CURVE ( 'NONE', #124197, #119064, #64724, .T. ) ;
#75858=EDGE_CURVE ( 'NONE', #122865, #1265, #77256, .T. ) ;
#75859=ORIENTED_EDGE ( 'NONE', *, *, #123228, .F. ) ;
#75860=ORIENTED_EDGE ( 'NONE', *, *, #58525, .T. ) ;
#75861=CARTESIAN_POINT ( 'NONE',  ( 7.099999999999928590, 12.50000000000000000, -4.330127018922201643 ) ) ;
#75862=AXIS2_PLACEMENT_3D ( 'NONE', #52010, #42858, #42185 ) ;
#75863=CARTESIAN_POINT ( 'NONE',  ( -4.150000000000024336, 2.500000000000000000, 2.065063509461097624 ) ) ;
#75864=ADVANCED_FACE ( 'NONE', ( #91231 ), #33364, .T. ) ;
#75865=CIRCLE ( 'NONE', #17361, 0.09999999999999982514 ) ;
#75866=CARTESIAN_POINT ( 'NONE',  ( -8.100000000000010303, 2.500000000000000000, 3.983716857408420964 ) ) ;
#75867=EDGE_LOOP ( 'NONE', ( #72997, #40020, #104628, #98054 ) ) ;
#75868=EDGE_LOOP ( 'NONE', ( #98010, #69586, #3517, #62704 ) ) ;
#75869=ADVANCED_FACE ( 'NONE', ( #39581 ), #20825, .T. ) ;
#75870=ORIENTED_EDGE ( 'NONE', *, *, #80285, .T. ) ;
#75871=EDGE_CURVE ( 'NONE', #99834, #92562, #78853, .T. ) ;
#75872=DIRECTION ( 'NONE',  ( 0.000000000000000000, 0.000000000000000000, -1.000000000000000000 ) ) ;
#75873=DIRECTION ( 'NONE',  ( 0.000000000000000000, 0.000000000000000000, -1.000000000000000000 ) ) ;
#75874=AXIS2_PLACEMENT_3D ( 'NONE', #32173, #81873, #80616 ) ;
#75875=AXIS2_PLACEMENT_3D ( 'NONE', #59382, #118914, #48243 ) ;
#75876=CARTESIAN_POINT ( 'NONE',  ( -4.600000000000028066, 2.500000000000000000, -5.022947341949754119 ) ) ;
#75877=CONICAL_SURFACE ( 'NONE', #9074, 0.09999999999999982514, 0.003490658503988666988 ) ;
#75879=EDGE_CURVE ( 'NONE', #83615, #122680, #21193, .T. ) ;
#75880=LINE ( 'NONE', #56236, #88764 ) ;
#75881=LINE ( 'NONE', #96162, #37711 ) ;
#75882=CARTESIAN_POINT ( 'NONE',  ( -9.350000000000006750, 2.500000000000000000, 2.511473670974873507 ) ) ;
#75883=AXIS2_PLACEMENT_3D ( 'NONE', #79107, #49650, #70552 ) ;
#75884=DIRECTION ( 'NONE',  ( 0.000000000000000000, 0.000000000000000000, 1.000000000000000000 ) ) ;
#75885=CARTESIAN_POINT ( 'NONE',  ( 14.39999999999989555, 2.500000000000000000, -0.4464101615137782142 ) ) ;
#75886=AXIS2_PLACEMENT_3D ( 'NONE', #48138, #959, #21240 ) ;
#75887=DIRECTION ( 'NONE',  ( 0.000000000000000000, 0.000000000000000000, 1.000000000000000000 ) ) ;
#75888=EDGE_CURVE ( 'NONE', #1361, #74448, #61121, .T. ) ;
#75889=CIRCLE ( 'NONE', #52914, 0.1000000000000000472 ) ;
#75890=ORIENTED_EDGE ( 'NONE', *, *, #25010, .F. ) ;
#75891=CARTESIAN_POINT ( 'NONE',  ( -4.150000000000028777, 12.50000000000000000, -5.802370205355749988 ) ) ;
#75893=EDGE_LOOP ( 'NONE', ( #103738, #90771 ) ) ;
#75894=CARTESIAN_POINT ( 'NONE',  ( 1.249999999999988898, 2.500000000000000000, -6.495190528383302464 ) ) ;
#75895=PLANE ( 'NONE',  #63652 ) ;
#75897=AXIS2_PLACEMENT_3D ( 'NONE', #102995, #13322, #6699 ) ;
#75898=DIRECTION ( 'NONE',  ( 0.000000000000000000, -0.000000000000000000, 1.000000000000000000 ) ) ;
#75899=DIRECTION ( 'NONE',  ( 0.000000000000000000, 1.000000000000000000, 0.000000000000000000 ) ) ;
#75900=CARTESIAN_POINT ( 'NONE',  ( 8.349999999999919709, 12.50000000000000000, 6.430097255199259010 ) ) ;
#75901=DIRECTION ( 'NONE',  ( 0.000000000000000000, 0.000000000000000000, 1.000000000000000000 ) ) ;
#75902=VERTEX_POINT ( 'NONE', #89929 ) ;
#75903=CARTESIAN_POINT ( 'NONE',  ( 2.949999999999946887, 12.50000000000000000, -2.165063509461101710 ) ) ;
#75904=VECTOR ( 'NONE', #51967, 1000.000000000000000 ) ;
#75905=FACE_OUTER_BOUND ( 'NONE', #70606, .T. ) ;
#75906=CIRCLE ( 'NONE', #34150, 0.06509327318403745899 ) ;
#75907=ORIENTED_EDGE ( 'NONE', *, *, #64061, .T. ) ;
#75908=AXIS2_PLACEMENT_3D ( 'NONE', #121497, #63244, #51504 ) ;
#75909=ORIENTED_EDGE ( 'NONE', *, *, #95607, .F. ) ;
#75910=VERTEX_POINT ( 'NONE', #20558 ) ;
#75911=ORIENTED_EDGE ( 'NONE', *, *, #49696, .T. ) ;
#75912=VECTOR ( 'NONE', #125550, 1000.000000000000000 ) ;
#75913=LINE ( 'NONE', #63532, #27404 ) ;
#75914=DIRECTION ( 'NONE',  ( 0.000000000000000000, 0.000000000000000000, 1.000000000000000000 ) ) ;
#75915=AXIS2_PLACEMENT_3D ( 'NONE', #92152, #91515, #32630 ) ;
#75916=AXIS2_PLACEMENT_3D ( 'NONE', #51086, #99537, #88393 ) ;
#75917=CARTESIAN_POINT ( 'NONE',  ( 6.249999999999932498, 12.50000000000000000, -5.802370205355749988 ) ) ;
#75918=CONICAL_SURFACE ( 'NONE', #605, 0.1000000000000000056, 0.003490658503988666988 ) ;
#75919=ADVANCED_FACE ( 'NONE', ( #69651 ), #50091, .T. ) ;
#75920=DIRECTION ( 'NONE',  ( 0.000000000000000000, -0.000000000000000000, 1.000000000000000000 ) ) ;
#75921=CARTESIAN_POINT ( 'NONE',  ( 2.299999999999949640, 2.500000000000000000, -0.3464101615137782364 ) ) ;
#75922=VERTEX_POINT ( 'NONE', #120690 ) ;
#75923=LINE ( 'NONE', #3961, #28579 ) ;
#75925=EDGE_CURVE ( 'NONE', #80146, #99999, #75198, .T. ) ;
#75926=ORIENTED_EDGE ( 'NONE', *, *, #70981, .F. ) ;
#75927=CIRCLE ( 'NONE', #19492, 0.06509327318403745899 ) ;
#75928=ORIENTED_EDGE ( 'NONE', *, *, #91991, .T. ) ;
#75929=VERTEX_POINT ( 'NONE', #31665 ) ;
#75930=DIRECTION ( 'NONE',  ( 0.000000000000000000, 1.000000000000000000, 0.000000000000000000 ) ) ;
#75931=CONICAL_SURFACE ( 'NONE', #36242, 0.1000000000000002554, 0.003490658503988666988 ) ;
#75932=PLANE ( 'NONE',  #46679 ) ;
#75933=DIRECTION ( 'NONE',  ( 0.000000000000000000, -0.000000000000000000, 1.000000000000000000 ) ) ;
#75934=ORIENTED_EDGE ( 'NONE', *, *, #27823, .F. ) ;
#75935=DIRECTION ( 'NONE',  ( 0.000000000000000000, 1.000000000000000000, 0.000000000000000000 ) ) ;
#75937=DIRECTION ( 'NONE',  ( -0.000000000000000000, 1.000000000000000000, -0.000000000000000000 ) ) ;
#75938=DIRECTION ( 'NONE',  ( -4.274815082592931898E-19, -0.9999939076577903929, -0.003490651415223739937 ) ) ;
#75939=CARTESIAN_POINT ( 'NONE',  ( 4.399999999999939071, 2.500000000000000000, 0.3464101615137736845 ) ) ;
#75940=ORIENTED_EDGE ( 'NONE', *, *, #61896, .T. ) ;
#75941=CARTESIAN_POINT ( 'NONE',  ( -7.900000000000014566, 2.500000000000000000, -3.637306695894650055 ) ) ;
#75942=ORIENTED_EDGE ( 'NONE', *, *, #93162, .F. ) ;
#75943=VERTEX_POINT ( 'NONE', #58557 ) ;
#75944=VECTOR ( 'NONE', #98737, 1000.000000000000000 ) ;
#75945=VERTEX_POINT ( 'NONE', #19243 ) ;
#75946=AXIS2_PLACEMENT_3D ( 'NONE', #31424, #62814, #81164 ) ;
#75947=DIRECTION ( 'NONE',  ( 0.000000000000000000, 1.000000000000000000, 0.000000000000000000 ) ) ;
#75948=FACE_BOUND ( 'NONE', #37411, .T. ) ;
#75949=CARTESIAN_POINT ( 'NONE',  ( 2.099999999999947686, 12.50000000000000000, 4.957854068765711553 ) ) ;
#75950=CARTESIAN_POINT ( 'NONE',  ( -5.600000000000020073, 2.500000000000000000, 3.983716857408420964 ) ) ;
#75951=FACE_OUTER_BOUND ( 'NONE', #86180, .T. ) ;
#75952=EDGE_CURVE ( 'NONE', #3331, #125340, #73052, .T. ) ;
#75953=CIRCLE ( 'NONE', #6982, 0.1000000000000000472 ) ;
#75954=VECTOR ( 'NONE', #17457, 1000.000000000000000 ) ;
#75955=AXIS2_PLACEMENT_3D ( 'NONE', #105939, #16242, #56182 ) ;
#75956=AXIS2_PLACEMENT_3D ( 'NONE', #10962, #81026, #24045 ) ;
#75957=CIRCLE ( 'NONE', #17462, 0.09999999999999982514 ) ;
#75958=EDGE_LOOP ( 'NONE', ( #119274, #54116, #22344, #29662 ) ) ;
#75959=DIRECTION ( 'NONE',  ( 0.000000000000000000, 0.000000000000000000, 1.000000000000000000 ) ) ;
#75960=CARTESIAN_POINT ( 'NONE',  ( 11.44999999999991047, 2.500000000000000000, -2.511473670974877948 ) ) ;
#75961=DIRECTION ( 'NONE',  ( 0.000000000000000000, 0.000000000000000000, -1.000000000000000000 ) ) ;
#75962=CARTESIAN_POINT ( 'NONE',  ( 17.50000000000000000, 2.500000000000000000, 0.000000000000000000 ) ) ;
#75963=VERTEX_POINT ( 'NONE', #51326 ) ;
#75965=AXIS2_PLACEMENT_3D ( 'NONE', #35378, #75286, #125661 ) ;
#75966=CARTESIAN_POINT ( 'NONE',  ( -3.750000000000025757, 2.500000000000000000, 1.572243186433545548 ) ) ;
#75967=CONICAL_SURFACE ( 'NONE', #55043, 0.1000000000000002554, 0.003490658503988666988 ) ;
#75968=CIRCLE ( 'NONE', #19537, 0.09999999999999982514 ) ;
#75969=DIRECTION ( 'NONE',  ( -0.000000000000000000, -1.000000000000000000, -0.000000000000000000 ) ) ;
#75970=CONICAL_SURFACE ( 'NONE', #59278, 0.1000000000000000056, 0.003490658503988666988 ) ;
#75971=ORIENTED_EDGE ( 'NONE', *, *, #121845, .T. ) ;
#75972=AXIS2_PLACEMENT_3D ( 'NONE', #95712, #104235, #15184 ) ;
#75973=EDGE_CURVE ( 'NONE', #129104, #97216, #110694, .T. ) ;
#75974=CARTESIAN_POINT ( 'NONE',  ( 5.849999999999935696, 12.50000000000000000, -6.495190528383302464 ) ) ;
#75975=EDGE_CURVE ( 'NONE', #50100, #123233, #81466, .T. ) ;
#75976=FACE_BOUND ( 'NONE', #33230, .T. ) ;
#75977=AXIS2_PLACEMENT_3D ( 'NONE', #106666, #37302, #36009 ) ;
#75978=CARTESIAN_POINT ( 'NONE',  ( -13.94999999999998863, 12.50000000000000000, 2.446380397790839822 ) ) ;
#75979=VERTEX_POINT ( 'NONE', #93176 ) ;
#75980=CARTESIAN_POINT ( 'NONE',  ( 9.549999999999915445, 12.50000000000000000, 6.495190528383297135 ) ) ;
#75981=CARTESIAN_POINT ( 'NONE',  ( 11.84999999999990727, 2.500000000000000000, -2.511473670974877948 ) ) ;
#75982=ADVANCED_FACE ( 'NONE', ( #54510 ), #18758, .T. ) ;
#75983=ORIENTED_EDGE ( 'NONE', *, *, #64645, .F. ) ;
#75984=EDGE_LOOP ( 'NONE', ( #124997, #28559 ) ) ;
#75985=ADVANCED_FACE ( 'NONE', ( #63057 ), #112771, .T. ) ;
#75987=EDGE_LOOP ( 'NONE', ( #79245, #76207, #87426, #5164 ) ) ;
#75988=CARTESIAN_POINT ( 'NONE',  ( 11.84999999999990372, 2.500000000000000000, 2.611473670974873151 ) ) ;
#75989=DIRECTION ( 'NONE',  ( 0.000000000000000000, 0.000000000000000000, 1.000000000000000000 ) ) ;
#75990=FACE_OUTER_BOUND ( 'NONE', #118192, .T. ) ;
#75991=FACE_OUTER_BOUND ( 'NONE', #78430, .T. ) ;
#75992=FACE_OUTER_BOUND ( 'NONE', #95186, .T. ) ;
#75994=VECTOR ( 'NONE', #123786, 1000.000000000000000 ) ;
#75996=ORIENTED_EDGE ( 'NONE', *, *, #118435, .T. ) ;
#75997=DIRECTION ( 'NONE',  ( 0.000000000000000000, -0.9999939076577903929, 0.003490651415223739937 ) ) ;
#75998=FACE_OUTER_BOUND ( 'NONE', #3611, .T. ) ;
#75999=DIRECTION ( 'NONE',  ( 0.000000000000000000, 0.000000000000000000, 1.000000000000000000 ) ) ;
#76000=DIRECTION ( 'NONE',  ( 0.000000000000000000, -0.000000000000000000, 1.000000000000000000 ) ) ;
#76001=EDGE_LOOP ( 'NONE', ( #20732, #108923 ) ) ;
#76002=VERTEX_POINT ( 'NONE', #12649 ) ;
#76003=FACE_BOUND ( 'NONE', #12127, .T. ) ;
#76004=ORIENTED_EDGE ( 'NONE', *, *, #64193, .F. ) ;
#76005=AXIS2_PLACEMENT_3D ( 'NONE', #84981, #7703, #77109 ) ;
#76007=CARTESIAN_POINT ( 'NONE',  ( -2.500000000000032419, 2.500000000000000000, -3.737306695894649700 ) ) ;
#76008=AXIS2_PLACEMENT_3D ( 'NONE', #93296, #25848, #4894 ) ;
#76009=ORIENTED_EDGE ( 'NONE', *, *, #37059, .F. ) ;
#76010=AXIS2_PLACEMENT_3D ( 'NONE', #34512, #104511, #6290 ) ;
#76011=PLANE ( 'NONE',  #38613 ) ;
#76012=LINE ( 'NONE', #115937, #5547 ) ;
#76013=VECTOR ( 'NONE', #62902, 1000.000000000000000 ) ;
#76014=EDGE_CURVE ( 'NONE', #21053, #16047, #16596, .T. ) ;
#76015=DIRECTION ( 'NONE',  ( 0.000000000000000000, 0.000000000000000000, 1.000000000000000000 ) ) ;
#76016=CARTESIAN_POINT ( 'NONE',  ( 14.14999999999989555, 2.500000000000000000, 2.265063509461097357 ) ) ;
#76017=ORIENTED_EDGE ( 'NONE', *, *, #120514, .F. ) ;
#76018=CARTESIAN_POINT ( 'NONE',  ( 3.099999999999943245, 2.500000000000000000, 3.883716857408420431 ) ) ;
#76019=CARTESIAN_POINT ( 'NONE',  ( -10.40000000000000213, 12.50000000000000000, -5.022947341949749678 ) ) ;
#76022=CIRCLE ( 'NONE', #21741, 0.1000000000000000056 ) ;
#76023=DIRECTION ( 'NONE',  ( 0.000000000000000000, 0.000000000000000000, 1.000000000000000000 ) ) ;
#76024=EDGE_CURVE ( 'NONE', #109299, #100844, #41800, .T. ) ;
#76025=EDGE_LOOP ( 'NONE', ( #30327, #57360, #45529, #110672 ) ) ;
#76026=ORIENTED_EDGE ( 'NONE', *, *, #23226, .F. ) ;
#76028=VECTOR ( 'NONE', #23815, 1000.000000000000000 ) ;
#76029=EDGE_LOOP ( 'NONE', ( #37598, #28187, #122511, #106203 ) ) ;
#76030=AXIS2_PLACEMENT_3D ( 'NONE', #12631, #72857, #2824 ) ;
#76031=CIRCLE ( 'NONE', #48858, 0.1000000000000002554 ) ;
#76032=DIRECTION ( 'NONE',  ( -0.000000000000000000, 1.000000000000000000, -0.000000000000000000 ) ) ;
#76034=EDGE_LOOP ( 'NONE', ( #114907, #71933 ) ) ;
#76035=ORIENTED_EDGE ( 'NONE', *, *, #9401, .T. ) ;
#76036=ORIENTED_EDGE ( 'NONE', *, *, #11933, .F. ) ;
#76037=AXIS2_PLACEMENT_3D ( 'NONE', #78917, #29170, #69069 ) ;
#76038=EDGE_CURVE ( 'NONE', #77490, #109874, #123235, .T. ) ;
#76039=DIRECTION ( 'NONE',  ( -0.000000000000000000, 1.000000000000000000, -0.000000000000000000 ) ) ;
#76040=ADVANCED_FACE ( 'NONE', ( #44059 ), #121983, .T. ) ;
#76041=VECTOR ( 'NONE', #76793, 1000.000000000000000 ) ;
#76044=EDGE_CURVE ( 'NONE', #87068, #8340, #100250, .T. ) ;
#76045=DIRECTION ( 'NONE',  ( -4.274815082592931898E-19, -0.9999939076577903929, -0.003490651415223739937 ) ) ;
#76046=DIRECTION ( 'NONE',  ( 0.000000000000000000, -0.9999939076577903929, 0.003490651415223739937 ) ) ;
#76047=CARTESIAN_POINT ( 'NONE',  ( 5.849999999999933920, 2.500000000000000000, 5.702370205355745014 ) ) ;
#76048=EDGE_LOOP ( 'NONE', ( #120808, #56086 ) ) ;
#76049=DIRECTION ( 'NONE',  ( 0.000000000000000000, 0.000000000000000000, 1.000000000000000000 ) ) ;
#76050=ADVANCED_FACE ( 'NONE', ( #33604 ), #52129, .T. ) ;
#76051=ORIENTED_EDGE ( 'NONE', *, *, #102189, .F. ) ;
#76052=EDGE_CURVE ( 'NONE', #59346, #110796, #108556, .T. ) ;
#76053=ORIENTED_EDGE ( 'NONE', *, *, #52192, .F. ) ;
#76054=ORIENTED_EDGE ( 'NONE', *, *, #119846, .T. ) ;
#76055=ORIENTED_EDGE ( 'NONE', *, *, #40424, .F. ) ;
#76056=CARTESIAN_POINT ( 'NONE',  ( -3.550000000000028244, 2.500000000000000000, -1.918653347947326004 ) ) ;
#76057=AXIS2_PLACEMENT_3D ( 'NONE', #82466, #113183, #33370 ) ;
#76058=ORIENTED_EDGE ( 'NONE', *, *, #89151, .T. ) ;
#76059=ORIENTED_EDGE ( 'NONE', *, *, #26242, .T. ) ;
#76060=CONICAL_SURFACE ( 'NONE', #69800, 0.1000000000000000472, 0.003490658503988666988 ) ;
#76061=DIRECTION ( 'NONE',  ( 0.000000000000000000, 1.000000000000000000, 0.000000000000000000 ) ) ;
#76062=AXIS2_PLACEMENT_3D ( 'NONE', #11182, #113096, #52897 ) ;
#76063=DIRECTION ( 'NONE',  ( 0.000000000000000000, 0.000000000000000000, -1.000000000000000000 ) ) ;
#76064=DIRECTION ( 'NONE',  ( -4.274815082592931898E-19, -0.9999939076577903929, -0.003490651415223739937 ) ) ;
#76065=DIRECTION ( 'NONE',  ( -4.274815082592931898E-19, -0.9999939076577903929, -0.003490651415223739937 ) ) ;
#76066=CONICAL_SURFACE ( 'NONE', #30112, 0.1000000000000000472, 0.003490658503988666988 ) ;
#76067=CONICAL_SURFACE ( 'NONE', #25886, 0.1000000000000000472, 0.003490658503988666988 ) ;
#76068=CARTESIAN_POINT ( 'NONE',  ( 0.8499999999999550138, 2.500000000000000000, -5.802370205355749988 ) ) ;
#76069=ORIENTED_EDGE ( 'NONE', *, *, #44369, .T. ) ;
#76070=CARTESIAN_POINT ( 'NONE',  ( 13.14999999999990088, 2.500000000000000000, 1.718653347947321386 ) ) ;
#76071=AXIS2_PLACEMENT_3D ( 'NONE', #72576, #32669, #82403 ) ;
#76072=CIRCLE ( 'NONE', #55145, 0.1000000000000000472 ) ;
#76073=ORIENTED_EDGE ( 'NONE', *, *, #6933, .T. ) ;
#76074=DIRECTION ( 'NONE',  ( 0.000000000000000000, -0.000000000000000000, 1.000000000000000000 ) ) ;
#76075=AXIS2_PLACEMENT_3D ( 'NONE', #65671, #97074, #5456 ) ;
#76076=EDGE_LOOP ( 'NONE', ( #109084, #63772, #66663, #54619 ) ) ;
#76077=CARTESIAN_POINT ( 'NONE',  ( 4.599999999999938360, 2.500000000000000000, -0.1000000000000022815 ) ) ;
#76078=EDGE_LOOP ( 'NONE', ( #70238, #128513 ) ) ;
#76079=CIRCLE ( 'NONE', #61429, 0.06509327318403745899 ) ;
#76080=ORIENTED_EDGE ( 'NONE', *, *, #86879, .F. ) ;
#76081=CARTESIAN_POINT ( 'NONE',  ( -11.69999999999999929, 2.500000000000000000, 1.734723475976807094E-15 ) ) ;
#76082=LINE ( 'NONE', #74797, #115327 ) ;
#76083=FACE_OUTER_BOUND ( 'NONE', #96462, .T. ) ;
#76084=EDGE_CURVE ( 'NONE', #129577, #121671, #125284, .T. ) ;
#76085=DIRECTION ( 'NONE',  ( 0.000000000000000000, 0.000000000000000000, -1.000000000000000000 ) ) ;
#76087=VERTEX_POINT ( 'NONE', #4753 ) ;
#76088=DIRECTION ( 'NONE',  ( 0.000000000000000000, -0.9999939076577903929, 0.003490651415223739937 ) ) ;
#76089=FACE_OUTER_BOUND ( 'NONE', #56225, .T. ) ;
#76090=CARTESIAN_POINT ( 'NONE',  ( 1.249999999999952038, 2.500000000000000000, -1.372243186433550033 ) ) ;
#76091=FACE_OUTER_BOUND ( 'NONE', #23665, .T. ) ;
#76092=CARTESIAN_POINT ( 'NONE',  ( -6.450000000000016165, 2.500000000000000000, 6.841600689897072485 ) ) ;
#76093=EDGE_CURVE ( 'NONE', #39360, #20166, #8377, .T. ) ;
#76094=ORIENTED_EDGE ( 'NONE', *, *, #36886, .T. ) ;
#76095=ORIENTED_EDGE ( 'NONE', *, *, #89151, .F. ) ;
#76096=CARTESIAN_POINT ( 'NONE',  ( -5.000000000000023093, 12.50000000000000000, 4.957854068765711553 ) ) ;
#76097=EDGE_LOOP ( 'NONE', ( #96995, #19786 ) ) ;
#76098=AXIS2_PLACEMENT_3D ( 'NONE', #2404, #112393, #82292 ) ;
#76099=DIRECTION ( 'NONE',  ( 0.000000000000000000, 1.000000000000000000, 0.000000000000000000 ) ) ;
#76100=DIRECTION ( 'NONE',  ( 0.000000000000000000, -0.000000000000000000, 1.000000000000000000 ) ) ;
#76101=AXIS2_PLACEMENT_3D ( 'NONE', #56317, #47810, #105437 ) ;
#76102=ORIENTED_EDGE ( 'NONE', *, *, #102189, .T. ) ;
#76104=CARTESIAN_POINT ( 'NONE',  ( 9.399999999999915090, 2.500000000000000000, -3.983716857408426293 ) ) ;
#76105=CARTESIAN_POINT ( 'NONE',  ( 13.34999999999989662, 2.500000000000000000, -2.065063509461102065 ) ) ;
#76106=DIRECTION ( 'NONE',  ( 0.000000000000000000, 0.000000000000000000, 1.000000000000000000 ) ) ;
#76107=AXIS2_PLACEMENT_3D ( 'NONE', #20764, #107852, #69869 ) ;
#76108=DIRECTION ( 'NONE',  ( 0.000000000000000000, -0.000000000000000000, 1.000000000000000000 ) ) ;
#76109=EDGE_LOOP ( 'NONE', ( #119300, #126884, #76167, #73112 ) ) ;
#76110=VECTOR ( 'NONE', #108230, 1000.000000000000000 ) ;
#76111=AXIS2_PLACEMENT_3D ( 'NONE', #23289, #52753, #94604 ) ;
#76112=CARTESIAN_POINT ( 'NONE',  ( -10.65000000000000391, 12.50000000000000000, -6.148780366869522673 ) ) ;
#76113=DIRECTION ( 'NONE',  ( 0.000000000000000000, -0.9999939076577903929, 0.003490651415223739937 ) ) ;
#76114=ORIENTED_EDGE ( 'NONE', *, *, #103961, .F. ) ;
#76115=DIRECTION ( 'NONE',  ( 0.000000000000000000, -0.000000000000000000, 1.000000000000000000 ) ) ;
#76116=DIRECTION ( 'NONE',  ( -0.000000000000000000, 1.000000000000000000, -0.000000000000000000 ) ) ;
#76117=LINE ( 'NONE', #95759, #23973 ) ;
#76118=EDGE_LOOP ( 'NONE', ( #122585, #30589, #106035, #57707 ) ) ;
#76119=CIRCLE ( 'NONE', #67796, 0.1000000000000002554 ) ;
#76120=AXIS2_PLACEMENT_3D ( 'NONE', #67877, #77689, #120215 ) ;
#76121=VECTOR ( 'NONE', #68236, 1000.000000000000000 ) ;
#76122=CARTESIAN_POINT ( 'NONE',  ( -12.09999999999999432, 2.500000000000000000, 3.637306695894644726 ) ) ;
#76123=VECTOR ( 'NONE', #34975, 1000.000000000000000 ) ;
#76124=ORIENTED_EDGE ( 'NONE', *, *, #53003, .T. ) ;
#76125=DIRECTION ( 'NONE',  ( -0.000000000000000000, 1.000000000000000000, -0.000000000000000000 ) ) ;
#76126=CARTESIAN_POINT ( 'NONE',  ( 6.249999999999932498, 2.500000000000000000, -5.702370205355749455 ) ) ;
#76127=DIRECTION ( 'NONE',  ( 0.000000000000000000, 0.000000000000000000, 1.000000000000000000 ) ) ;
#76129=EDGE_LOOP ( 'NONE', ( #109451, #89135, #47250, #11880 ) ) ;
#76130=EDGE_CURVE ( 'NONE', #76377, #2854, #106582, .T. ) ;
#76131=CARTESIAN_POINT ( 'NONE',  ( -4.350000000000027178, 2.500000000000000000, -6.148780366869526226 ) ) ;
#76132=DIRECTION ( 'NONE',  ( 0.000000000000000000, -0.000000000000000000, 1.000000000000000000 ) ) ;
#76133=ORIENTED_EDGE ( 'NONE', *, *, #24452, .F. ) ;
#76134=ADVANCED_FACE ( 'NONE', ( #112163 ), #58578, .T. ) ;
#76135=EDGE_CURVE ( 'NONE', #33970, #18481, #21863, .T. ) ;
#76136=ORIENTED_EDGE ( 'NONE', *, *, #58988, .T. ) ;
#76137=CARTESIAN_POINT ( 'NONE',  ( 5.849999999999933031, 2.500000000000000000, -1.572243186433550211 ) ) ;
#76138=ORIENTED_EDGE ( 'NONE', *, *, #55909, .F. ) ;
#76139=CARTESIAN_POINT ( 'NONE',  ( 4.799999999999934097, 12.50000000000000000, 4.676537180435972552 ) ) ;
#76140=DIRECTION ( 'NONE',  ( 0.000000000000000000, -0.000000000000000000, 1.000000000000000000 ) ) ;
#76141=EDGE_CURVE ( 'NONE', #112646, #127507, #104532, .T. ) ;
#76142=VECTOR ( 'NONE', #97325, 1000.000000000000000 ) ;
#76143=ADVANCED_FACE ( 'NONE', ( #51962 ), #14622, .T. ) ;
#76144=CIRCLE ( 'NONE', #46907, 0.06509327318403745899 ) ;
#76145=CIRCLE ( 'NONE', #105392, 0.1000000000000000472 ) ;
#76146=ORIENTED_EDGE ( 'NONE', *, *, #45395, .F. ) ;
#76147=ADVANCED_FACE ( 'NONE', ( #95101 ), #10443, .T. ) ;
#76148=DIRECTION ( 'NONE',  ( 0.000000000000000000, 1.000000000000000000, 0.000000000000000000 ) ) ;
#76149=CARTESIAN_POINT ( 'NONE',  ( 14.14999999999989377, 2.500000000000000000, -1.472243186433550122 ) ) ;
#76150=ORIENTED_EDGE ( 'NONE', *, *, #43661, .F. ) ;
#76151=PLANE ( 'NONE',  #19641 ) ;
#76152=AXIS2_PLACEMENT_3D ( 'NONE', #23479, #40066, #111870 ) ;
#76153=CARTESIAN_POINT ( 'NONE',  ( -0.8000000000000376810, 2.500000000000000000, -4.330127018922201643 ) ) ;
#76154=AXIS2_PLACEMENT_3D ( 'NONE', #41015, #120837, #10239 ) ;
#76155=AXIS2_PLACEMENT_3D ( 'NONE', #75445, #113447, #55816 ) ;
#76156=AXIS2_PLACEMENT_3D ( 'NONE', #100202, #88427, #49189 ) ;
#76157=CARTESIAN_POINT ( 'NONE',  ( 17.34779069867702361, -2.317761454549422506, -4.873653559264009338 ) ) ;
#76158=DIRECTION ( 'NONE',  ( 0.000000000000000000, -0.9999939076577903929, 0.003490651415223739937 ) ) ;
#76159=DIRECTION ( 'NONE',  ( 0.000000000000000000, 1.000000000000000000, 0.000000000000000000 ) ) ;
#76160=FACE_OUTER_BOUND ( 'NONE', #50101, .T. ) ;
#76161=AXIS2_PLACEMENT_3D ( 'NONE', #77700, #8959, #126820 ) ;
#76162=AXIS2_PLACEMENT_3D ( 'NONE', #50312, #71229, #52890 ) ;
#76163=AXIS2_PLACEMENT_3D ( 'NONE', #90459, #32224, #111385 ) ;
#76164=ORIENTED_EDGE ( 'NONE', *, *, #22269, .F. ) ;
#76165=ORIENTED_EDGE ( 'NONE', *, *, #37875, .T. ) ;
#76166=ORIENTED_EDGE ( 'NONE', *, *, #47971, .F. ) ;
#76167=ORIENTED_EDGE ( 'NONE', *, *, #119498, .T. ) ;
#76168=DIRECTION ( 'NONE',  ( 0.000000000000000000, 1.000000000000000000, 0.000000000000000000 ) ) ;
#76169=DIRECTION ( 'NONE',  ( 0.000000000000000000, 0.000000000000000000, 1.000000000000000000 ) ) ;
#76170=AXIS2_PLACEMENT_3D ( 'NONE', #26811, #87011, #75901 ) ;
#76171=DIRECTION ( 'NONE',  ( 0.000000000000000000, 0.000000000000000000, -1.000000000000000000 ) ) ;
#76172=ORIENTED_EDGE ( 'NONE', *, *, #21456, .T. ) ;
#76173=FACE_BOUND ( 'NONE', #108806, .T. ) ;
#76174=DIRECTION ( 'NONE',  ( -0.000000000000000000, -1.000000000000000000, -0.000000000000000000 ) ) ;
#76175=CARTESIAN_POINT ( 'NONE',  ( -3.950000000000025491, 12.50000000000000000, 6.148780366869520897 ) ) ;
#76176=DIRECTION ( 'NONE',  ( 0.000000000000000000, 1.000000000000000000, 0.000000000000000000 ) ) ;
#76177=DIRECTION ( 'NONE',  ( -0.000000000000000000, -1.000000000000000000, -0.000000000000000000 ) ) ;
#76178=CARTESIAN_POINT ( 'NONE',  ( 16.87640210516308770, -2.500000000000000000, -4.436424697255247906 ) ) ;
#76179=DIRECTION ( 'NONE',  ( 0.000000000000000000, 0.000000000000000000, -1.000000000000000000 ) ) ;
#76181=FACE_OUTER_BOUND ( 'NONE', #109557, .T. ) ;
#76182=CARTESIAN_POINT ( 'NONE',  ( 10.19999999999991225, 2.500000000000000000, 4.083716857408420609 ) ) ;
#76183=DIRECTION ( 'NONE',  ( 0.000000000000000000, 0.000000000000000000, 1.000000000000000000 ) ) ;
#76184=CIRCLE ( 'NONE', #92918, 0.1000000000000000472 ) ;
#76185=FACE_OUTER_BOUND ( 'NONE', #15633, .T. ) ;
#76186=VERTEX_POINT ( 'NONE', #104896 ) ;
#76187=EDGE_LOOP ( 'NONE', ( #97016, #27765 ) ) ;
#76188=ORIENTED_EDGE ( 'NONE', *, *, #13944, .F. ) ;
#76189=ORIENTED_EDGE ( 'NONE', *, *, #89742, .F. ) ;
#76190=CARTESIAN_POINT ( 'NONE',  ( 6.049999999999934097, 2.500000000000000000, -2.611473670974877592 ) ) ;
#76191=EDGE_LOOP ( 'NONE', ( #109774, #119030 ) ) ;
#76192=EDGE_CURVE ( 'NONE', #56136, #52780, #87793, .T. ) ;
#76193=CARTESIAN_POINT ( 'NONE',  ( 10.59999999999990905, 12.50000000000000000, -4.676537180435978769 ) ) ;
#76194=EDGE_CURVE ( 'NONE', #85461, #116268, #73145, .T. ) ;
#76195=ORIENTED_EDGE ( 'NONE', *, *, #23880, .F. ) ;
#76196=ORIENTED_EDGE ( 'NONE', *, *, #5205, .T. ) ;
#76197=ADVANCED_FACE ( 'NONE', ( #36187 ), #83618, .T. ) ;
#76198=CARTESIAN_POINT ( 'NONE',  ( -10.65000000000000213, 12.50000000000000000, 2.576566944158910744 ) ) ;
#76199=AXIS2_PLACEMENT_3D ( 'NONE', #27219, #65193, #115588 ) ;
#76200=AXIS2_PLACEMENT_3D ( 'NONE', #126861, #26085, #116374 ) ;
#76201=DIRECTION ( 'NONE',  ( -0.000000000000000000, -1.000000000000000000, -0.000000000000000000 ) ) ;
#76202=CARTESIAN_POINT ( 'NONE',  ( 3.549999999999942979, 2.500000000000000000, 1.918653347947321564 ) ) ;
#76203=CARTESIAN_POINT ( 'NONE',  ( 5.399999999999932854, 12.50000000000000000, 3.702399969078682407 ) ) ;
#76204=EDGE_CURVE ( 'NONE', #18883, #59390, #64816, .T. ) ;
#76205=DIRECTION ( 'NONE',  ( 0.000000000000000000, -0.000000000000000000, 1.000000000000000000 ) ) ;
#76206=EDGE_CURVE ( 'NONE', #10596, #15192, #117027, .T. ) ;
#76207=ORIENTED_EDGE ( 'NONE', *, *, #18954, .T. ) ;
#76208=ADVANCED_FACE ( 'NONE', ( #86555 ), #17809, .T. ) ;
#76209=EDGE_CURVE ( 'NONE', #105930, #123334, #15214, .T. ) ;
#76210=ORIENTED_EDGE ( 'NONE', *, *, #88142, .F. ) ;
#76211=CIRCLE ( 'NONE', #80321, 0.06509327318403745899 ) ;
#76212=EDGE_CURVE ( 'NONE', #7922, #108419, #48104, .T. ) ;
#76213=ORIENTED_EDGE ( 'NONE', *, *, #14245, .T. ) ;
#76214=ORIENTED_EDGE ( 'NONE', *, *, #67889, .F. ) ;
#76215=CIRCLE ( 'NONE', #120123, 0.06509327318403745899 ) ;
#76216=CARTESIAN_POINT ( 'NONE',  ( 13.09999999999990195, 2.500000000000000000, -4.776537180435978414 ) ) ;
#76217=EDGE_LOOP ( 'NONE', ( #43958, #35643 ) ) ;
#76218=EDGE_LOOP ( 'NONE', ( #3073, #62594, #120415, #78804 ) ) ;
#76219=EDGE_CURVE ( 'NONE', #96705, #38043, #33450, .T. ) ;
#76220=DIRECTION ( 'NONE',  ( 0.000000000000000000, 0.000000000000000000, 1.000000000000000000 ) ) ;
#76221=CARTESIAN_POINT ( 'NONE',  ( 11.24999999999990941, 2.500000000000000000, -1.572243186433550211 ) ) ;
#76222=VECTOR ( 'NONE', #70662, 1000.000000000000000 ) ;
#76223=DIRECTION ( 'NONE',  ( 0.000000000000000000, 0.000000000000000000, 1.000000000000000000 ) ) ;
#76224=CIRCLE ( 'NONE', #107512, 0.06509327318403745899 ) ;
#76226=DIRECTION ( 'NONE',  ( -4.274815082592931898E-19, -0.9999939076577903929, -0.003490651415223739937 ) ) ;
#76227=CARTESIAN_POINT ( 'NONE',  ( -2.100000000000033840, 12.50000000000000000, 5.022947341949748790 ) ) ;
#76228=AXIS2_PLACEMENT_3D ( 'NONE', #64881, #84537, #124469 ) ;
#76229=ORIENTED_EDGE ( 'NONE', *, *, #2864, .T. ) ;
#76230=CIRCLE ( 'NONE', #19790, 0.1000000000000002554 ) ;
#76232=ORIENTED_EDGE ( 'NONE', *, *, #106890, .T. ) ;
#76233=DIRECTION ( 'NONE',  ( 0.000000000000000000, 1.000000000000000000, 0.000000000000000000 ) ) ;
#76234=ORIENTED_EDGE ( 'NONE', *, *, #96889, .T. ) ;
#76235=FACE_OUTER_BOUND ( 'NONE', #65954, .T. ) ;
#76236=DIRECTION ( 'NONE',  ( -0.000000000000000000, 1.000000000000000000, -0.000000000000000000 ) ) ;
#76237=EDGE_LOOP ( 'NONE', ( #11305, #97922, #31907, #472 ) ) ;
#76238=CARTESIAN_POINT ( 'NONE',  ( 3.749999999999940492, 12.50000000000000000, 5.737276932171707422 ) ) ;
#76239=LINE ( 'NONE', #106336, #85647 ) ;
#76240=ORIENTED_EDGE ( 'NONE', *, *, #14547, .T. ) ;
#76241=AXIS2_PLACEMENT_3D ( 'NONE', #1210, #9746, #11672 ) ;
#76242=CONICAL_SURFACE ( 'NONE', #11482, 0.09999999999999982514, 0.003490658503988666988 ) ;
#76243=DIRECTION ( 'NONE',  ( 0.000000000000000000, 0.000000000000000000, -1.000000000000000000 ) ) ;
#76244=VERTEX_POINT ( 'NONE', #107495 ) ;
#76245=CONICAL_SURFACE ( 'NONE', #49068, 0.1000000000000002554, 0.003490658503988666988 ) ;
#76246=VECTOR ( 'NONE', #55420, 1000.000000000000000 ) ;
#76247=EDGE_LOOP ( 'NONE', ( #126020, #116760, #48057, #31539 ) ) ;
#76248=DIRECTION ( 'NONE',  ( 0.000000000000000000, 0.000000000000000000, 1.000000000000000000 ) ) ;
#76249=DIRECTION ( 'NONE',  ( -4.274815082592931898E-19, -0.9999939076577903929, -0.003490651415223739937 ) ) ;
#76251=LINE ( 'NONE', #36970, #13616 ) ;
#76252=VECTOR ( 'NONE', #4380, 1000.000000000000000 ) ;
#76253=CARTESIAN_POINT ( 'NONE',  ( -10.80000000000000071, 2.500000000000000000, 4.430127018922196847 ) ) ;
#76254=EDGE_CURVE ( 'NONE', #28910, #24882, #94072, .T. ) ;
#76255=AXIS2_PLACEMENT_3D ( 'NONE', #62190, #32736, #92263 ) ;
#76256=CONICAL_SURFACE ( 'NONE', #84651, 0.09999999999999982514, 0.003490658503988666988 ) ;
#76257=DIRECTION ( 'NONE',  ( 0.000000000000000000, 1.000000000000000000, 0.000000000000000000 ) ) ;
#76259=ORIENTED_EDGE ( 'NONE', *, *, #51792, .T. ) ;
#76260=VECTOR ( 'NONE', #112305, 1000.000000000000000 ) ;
#76261=CARTESIAN_POINT ( 'NONE',  ( -9.200000000000006395, 2.500000000000000000, 0.09999999999999761857 ) ) ;
#76262=ORIENTED_EDGE ( 'NONE', *, *, #97036, .F. ) ;
#76263=AXIS2_PLACEMENT_3D ( 'NONE', #40360, #10851, #101202 ) ;
#76264=DIRECTION ( 'NONE',  ( 0.000000000000000000, 0.000000000000000000, 1.000000000000000000 ) ) ;
#76265=CARTESIAN_POINT ( 'NONE',  ( -15.19999999999998153, 12.50000000000000000, -0.3464101615137759604 ) ) ;
#76266=DIRECTION ( 'NONE',  ( -4.274815082592931898E-19, -0.9999939076577903929, -0.003490651415223739937 ) ) ;
#76267=ORIENTED_EDGE ( 'NONE', *, *, #112797, .F. ) ;
#76268=CARTESIAN_POINT ( 'NONE',  ( 14.14999999999989200, 2.500000000000000000, -2.165063509461101710 ) ) ;
#76269=DIRECTION ( 'NONE',  ( 0.000000000000000000, 0.000000000000000000, 1.000000000000000000 ) ) ;
#76270=AXIS2_PLACEMENT_3D ( 'NONE', #38849, #20471, #120596 ) ;
#76271=EDGE_LOOP ( 'NONE', ( #21539, #31042, #49374, #67532 ) ) ;
#76272=DIRECTION ( 'NONE',  ( -0.000000000000000000, -1.000000000000000000, -0.000000000000000000 ) ) ;
#76273=EDGE_LOOP ( 'NONE', ( #71256, #39136, #124907, #27990 ) ) ;
#76274=EDGE_LOOP ( 'NONE', ( #53639, #22618 ) ) ;
#76275=FACE_OUTER_BOUND ( 'NONE', #15410, .T. ) ;
#76276=VERTEX_POINT ( 'NONE', #87192 ) ;
#76277=DIRECTION ( 'NONE',  ( -0.000000000000000000, 1.000000000000000000, -0.000000000000000000 ) ) ;
#76278=DIRECTION ( 'NONE',  ( 0.000000000000000000, 0.000000000000000000, -1.000000000000000000 ) ) ;
#76279=AXIS2_PLACEMENT_3D ( 'NONE', #25134, #4836, #123974 ) ;
#76280=DIRECTION ( 'NONE',  ( 0.000000000000000000, 0.000000000000000000, 1.000000000000000000 ) ) ;
#76281=AXIS2_PLACEMENT_3D ( 'NONE', #11582, #32542, #63261 ) ;
#76282=ORIENTED_EDGE ( 'NONE', *, *, #49578, .T. ) ;
#76283=ADVANCED_FACE ( 'NONE', ( #87834 ), #55814, .T. ) ;
#76284=FACE_BOUND ( 'NONE', #71033, .T. ) ;
#76285=DIRECTION ( 'NONE',  ( 0.000000000000000000, 0.000000000000000000, -1.000000000000000000 ) ) ;
#76286=EDGE_LOOP ( 'NONE', ( #4658, #94828 ) ) ;
#76287=DIRECTION ( 'NONE',  ( 0.000000000000000000, 0.000000000000000000, 1.000000000000000000 ) ) ;
#76288=CARTESIAN_POINT ( 'NONE',  ( -9.999999999999969802, 12.50000000000000000, -2.276824562219559311E-15 ) ) ;
#76289=EDGE_CURVE ( 'NONE', #61621, #56423, #27166, .T. ) ;
#76290=ORIENTED_EDGE ( 'NONE', *, *, #75410, .T. ) ;
#76291=ORIENTED_EDGE ( 'NONE', *, *, #85880, .F. ) ;
#76292=CIRCLE ( 'NONE', #78464, 0.1000000000000002554 ) ;
#76293=VERTEX_POINT ( 'NONE', #55174 ) ;
#76294=DIRECTION ( 'NONE',  ( 0.000000000000000000, 1.000000000000000000, 0.000000000000000000 ) ) ;
#76295=DIRECTION ( 'NONE',  ( -0.000000000000000000, -1.000000000000000000, -0.000000000000000000 ) ) ;
#76296=EDGE_CURVE ( 'NONE', #109309, #77648, #25106, .T. ) ;
#76297=ADVANCED_FACE ( 'NONE', ( #116015 ), #27620, .T. ) ;
#76298=CARTESIAN_POINT ( 'NONE',  ( -11.25000000000000000, 2.500000000000000000, 7.188010851410848723 ) ) ;
#76299=EDGE_CURVE ( 'NONE', #58714, #34192, #56445, .T. ) ;
#76300=FACE_BOUND ( 'NONE', #104139, .T. ) ;
#76301=EDGE_LOOP ( 'NONE', ( #15415, #114626, #35809, #112462 ) ) ;
#76302=EDGE_CURVE ( 'NONE', #121670, #57274, #75280, .T. ) ;
#76304=ADVANCED_FACE ( 'NONE', ( #119240 ), #112856, .T. ) ;
#76305=DIRECTION ( 'NONE',  ( 0.000000000000000000, 1.000000000000000000, 0.000000000000000000 ) ) ;
#76306=CARTESIAN_POINT ( 'NONE',  ( 9.799999999999918998, 2.500000000000000000, -0.4464101615137782142 ) ) ;
#76307=CIRCLE ( 'NONE', #111905, 0.06509327318403745899 ) ;
#76308=CARTESIAN_POINT ( 'NONE',  ( -3.150000000000030109, 2.500000000000000000, 1.918653347947321564 ) ) ;
#76309=CIRCLE ( 'NONE', #126489, 0.1000000000000002554 ) ;
#76310=FACE_OUTER_BOUND ( 'NONE', #12978, .T. ) ;
#76311=CARTESIAN_POINT ( 'NONE',  ( 7.099999999999926814, 2.500000000000000000, -2.276824562219559311E-15 ) ) ;
#76312=EDGE_CURVE ( 'NONE', #103846, #87255, #105, .T. ) ;
#76313=CARTESIAN_POINT ( 'NONE',  ( -8.150000000000012790, 2.500000000000000000, -2.411473670974877859 ) ) ;
#76314=DIRECTION ( 'NONE',  ( -0.000000000000000000, 1.000000000000000000, -0.000000000000000000 ) ) ;
#76315=EDGE_CURVE ( 'NONE', #57789, #31107, #119113, .T. ) ;
#76316=CARTESIAN_POINT ( 'NONE',  ( 14.14999999999989377, 2.500000000000000000, -1.472243186433550122 ) ) ;
#76317=ORIENTED_EDGE ( 'NONE', *, *, #97136, .T. ) ;
#76318=EDGE_LOOP ( 'NONE', ( #76920, #27045 ) ) ;
#76319=ORIENTED_EDGE ( 'NONE', *, *, #10800, .F. ) ;
#76320=VERTEX_POINT ( 'NONE', #19764 ) ;
#76321=ORIENTED_EDGE ( 'NONE', *, *, #85629, .T. ) ;
#76323=CARTESIAN_POINT ( 'NONE',  ( 4.349999999999941025, 2.500000000000000000, -1.918653347947326004 ) ) ;
#76324=VERTEX_POINT ( 'NONE', #69487 ) ;
#76325=FACE_BOUND ( 'NONE', #22613, .T. ) ;
#76326=CIRCLE ( 'NONE', #109871, 0.06509327318403745899 ) ;
#76327=CARTESIAN_POINT ( 'NONE',  ( -8.100000000000013856, 2.500000000000000000, -3.983716857408426293 ) ) ;
#76328=AXIS2_PLACEMENT_3D ( 'NONE', #50110, #61200, #89997 ) ;
#76329=DIRECTION ( 'NONE',  ( -0.000000000000000000, 1.000000000000000000, -0.000000000000000000 ) ) ;
#76330=AXIS2_PLACEMENT_3D ( 'NONE', #110219, #127288, #87332 ) ;
#76331=AXIS2_PLACEMENT_3D ( 'NONE', #52517, #92442, #2774 ) ;
#76332=CARTESIAN_POINT ( 'NONE',  ( -13.34999999999999076, 2.500000000000000000, 2.857883832488652853 ) ) ;
#76333=DIRECTION ( 'NONE',  ( -0.000000000000000000, -1.000000000000000000, -0.000000000000000000 ) ) ;
#76334=DIRECTION ( 'NONE',  ( 0.000000000000000000, 0.000000000000000000, 1.000000000000000000 ) ) ;
#76335=EDGE_LOOP ( 'NONE', ( #110949, #41377, #77410, #11400 ) ) ;
#76337=AXIS2_PLACEMENT_3D ( 'NONE', #56078, #126772, #37108 ) ;
#76338=EDGE_LOOP ( 'NONE', ( #116866, #47431 ) ) ;
#76340=AXIS2_PLACEMENT_3D ( 'NONE', #111472, #51296, #883 ) ;
#76341=ORIENTED_EDGE ( 'NONE', *, *, #18242, .T. ) ;
#76342=ORIENTED_EDGE ( 'NONE', *, *, #67132, .T. ) ;
#76343=CARTESIAN_POINT ( 'NONE',  ( 5.599999999999934808, 2.500000000000000000, -3.983716857408426293 ) ) ;
#76344=AXIS2_PLACEMENT_3D ( 'NONE', #37151, #78368, #37785 ) ;
#76345=DIRECTION ( 'NONE',  ( 0.000000000000000000, 0.000000000000000000, -1.000000000000000000 ) ) ;
#76346=DIRECTION ( 'NONE',  ( 0.000000000000000000, -0.9999939076577903929, 0.003490651415223739937 ) ) ;
#76347=ORIENTED_EDGE ( 'NONE', *, *, #56068, .T. ) ;
#76348=CARTESIAN_POINT ( 'NONE',  ( 15.83209681635555022, 2.499999999999999556, -5.404881881984137770 ) ) ;
#76349=EDGE_CURVE ( 'NONE', #10759, #28226, #68851, .T. ) ;
#76350=CONICAL_SURFACE ( 'NONE', #47115, 0.1000000000000000056, 0.003490658503988666988 ) ;
#76351=AXIS2_PLACEMENT_3D ( 'NONE', #33672, #63784, #21930 ) ;
#76352=LINE ( 'NONE', #78297, #103430 ) ;
#76354=DIRECTION ( 'NONE',  ( 0.000000000000000000, 0.000000000000000000, 1.000000000000000000 ) ) ;
#76357=AXIS2_PLACEMENT_3D ( 'NONE', #2325, #24405, #42282 ) ;
#76358=CARTESIAN_POINT ( 'NONE',  ( 12.29999999999990656, 12.50000000000000000, 3.983716857408420964 ) ) ;
#76359=EDGE_CURVE ( 'NONE', #56076, #126920, #18845, .T. ) ;
#76360=EDGE_LOOP ( 'NONE', ( #75749, #48760, #64707, #14837 ) ) ;
#76361=CARTESIAN_POINT ( 'NONE',  ( 1.649999999999951505, 2.500000000000000000, 2.857883832488649301 ) ) ;
#76362=EDGE_CURVE ( 'NONE', #12477, #79083, #79419, .T. ) ;
#76363=VERTEX_POINT ( 'NONE', #109425 ) ;
#76364=ADVANCED_FACE ( 'NONE', ( #91071 ), #22976, .T. ) ;
#76365=ORIENTED_EDGE ( 'NONE', *, *, #126441, .T. ) ;
#76367=DIRECTION ( 'NONE',  ( 0.000000000000000000, 1.000000000000000000, 0.000000000000000000 ) ) ;
#76368=PLANE ( 'NONE',  #23763 ) ;
#76369=CIRCLE ( 'NONE', #47129, 0.1000000000000002554 ) ;
#76370=EDGE_LOOP ( 'NONE', ( #97623, #106783 ) ) ;
#76372=EDGE_LOOP ( 'NONE', ( #17024, #8261, #32594, #8657 ) ) ;
#76373=DIRECTION ( 'NONE',  ( 0.000000000000000000, 1.000000000000000000, 0.000000000000000000 ) ) ;
#76374=CARTESIAN_POINT ( 'NONE',  ( -7.500000000000015099, 2.500000000000000000, -5.122947341949753763 ) ) ;
#76375=DIRECTION ( 'NONE',  ( 0.000000000000000000, 0.000000000000000000, 1.000000000000000000 ) ) ;
#76376=ORIENTED_EDGE ( 'NONE', *, *, #118878, .T. ) ;
#76377=VERTEX_POINT ( 'NONE', #49238 ) ;
#76378=DIRECTION ( 'NONE',  ( 0.000000000000000000, 1.000000000000000000, 0.000000000000000000 ) ) ;
#76379=AXIS2_PLACEMENT_3D ( 'NONE', #54428, #74079, #36094 ) ;
#76380=CIRCLE ( 'NONE', #53395, 0.09999999999999982514 ) ;
#76381=ORIENTED_EDGE ( 'NONE', *, *, #62462, .T. ) ;
#76382=DIRECTION ( 'NONE',  ( -0.000000000000000000, 1.000000000000000000, -0.000000000000000000 ) ) ;
#76383=CIRCLE ( 'NONE', #40897, 0.06509327318403745899 ) ;
#76384=CARTESIAN_POINT ( 'NONE',  ( -11.04999999999999893, 2.500000000000000000, 1.718653347947321386 ) ) ;
#76385=ORIENTED_EDGE ( 'NONE', *, *, #124751, .T. ) ;
#76386=DIRECTION ( 'NONE',  ( 0.000000000000000000, 0.000000000000000000, -1.000000000000000000 ) ) ;
#76388=CARTESIAN_POINT ( 'NONE',  ( -0.6000000000000323963, 2.500000000000000000, -0.2464101615137759549 ) ) ;
#76389=EDGE_CURVE ( 'NONE', #64274, #40995, #54356, .T. ) ;
#76390=DIRECTION ( 'NONE',  ( -0.000000000000000000, 1.000000000000000000, -0.000000000000000000 ) ) ;
#76391=ORIENTED_EDGE ( 'NONE', *, *, #119909, .T. ) ;
#76392=CIRCLE ( 'NONE', #3233, 0.1000000000000002554 ) ;
#76393=DIRECTION ( 'NONE',  ( 0.000000000000000000, 0.000000000000000000, -1.000000000000000000 ) ) ;
#76394=DIRECTION ( 'NONE',  ( 0.000000000000000000, 0.000000000000000000, 1.000000000000000000 ) ) ;
#76395=VECTOR ( 'NONE', #27363, 1000.000000000000000 ) ;
#76396=ORIENTED_EDGE ( 'NONE', *, *, #49037, .T. ) ;
#76397=ORIENTED_EDGE ( 'NONE', *, *, #54705, .T. ) ;
#76399=DIRECTION ( 'NONE',  ( -0.000000000000000000, -1.000000000000000000, -0.000000000000000000 ) ) ;
#76400=DIRECTION ( 'NONE',  ( 0.000000000000000000, -0.000000000000000000, 1.000000000000000000 ) ) ;
#76402=DIRECTION ( 'NONE',  ( 0.000000000000000000, 0.000000000000000000, 1.000000000000000000 ) ) ;
#76403=DIRECTION ( 'NONE',  ( 0.000000000000000000, 1.000000000000000000, 0.000000000000000000 ) ) ;
#76404=AXIS2_PLACEMENT_3D ( 'NONE', #95302, #5605, #125404 ) ;
#76405=AXIS2_PLACEMENT_3D ( 'NONE', #53959, #44133, #115418 ) ;
#76406=CARTESIAN_POINT ( 'NONE',  ( 17.46754056294894752, 1.506946016794848742, -5.249106941592859066 ) ) ;
#76407=ADVANCED_FACE ( 'NONE', ( #99616 ), #48191, .T. ) ;
#76408=DIRECTION ( 'NONE',  ( 0.000000000000000000, 1.000000000000000000, 0.000000000000000000 ) ) ;
#76409=CARTESIAN_POINT ( 'NONE',  ( 11.64999999999990798, 2.500000000000000000, -2.757883832488654097 ) ) ;
#76410=DIRECTION ( 'NONE',  ( 0.000000000000000000, -0.9999939076577903929, 0.003490651415223739937 ) ) ;
#76411=EDGE_LOOP ( 'NONE', ( #22686, #30975 ) ) ;
#76413=ORIENTED_EDGE ( 'NONE', *, *, #45277, .F. ) ;
#76414=DIRECTION ( 'NONE',  ( 0.000000000000000000, -0.000000000000000000, 1.000000000000000000 ) ) ;
#76415=EDGE_LOOP ( 'NONE', ( #112722, #94634 ) ) ;
#76416=EDGE_CURVE ( 'NONE', #56250, #112093, #87877, .T. ) ;
#76417=LINE ( 'NONE', #105224, #87535 ) ;
#76418=CONICAL_SURFACE ( 'NONE', #1195, 0.09999999999999982514, 0.003490658503988666988 ) ;
#76419=CARTESIAN_POINT ( 'NONE',  ( -14.34999999999998543, 2.500000000000000000, 1.818653347947325472 ) ) ;
#76420=DIRECTION ( 'NONE',  ( -0.000000000000000000, -1.000000000000000000, -0.000000000000000000 ) ) ;
#76421=ORIENTED_EDGE ( 'NONE', *, *, #14659, .T. ) ;
#76422=DIRECTION ( 'NONE',  ( 0.000000000000000000, 0.000000000000000000, 1.000000000000000000 ) ) ;
#76423=CIRCLE ( 'NONE', #5397, 0.1000000000000002554 ) ;
#76425=PLANE ( 'NONE',  #27174 ) ;
#76426=ORIENTED_EDGE ( 'NONE', *, *, #64153, .F. ) ;
#76427=CARTESIAN_POINT ( 'NONE',  ( -10.20000000000000284, 2.500000000000000000, 4.083716857408421497 ) ) ;
#76428=EDGE_LOOP ( 'NONE', ( #63671, #37105 ) ) ;
#76429=EDGE_LOOP ( 'NONE', ( #75486, #34905 ) ) ;
#76430=VERTEX_POINT ( 'NONE', #60343 ) ;
#76431=VERTEX_POINT ( 'NONE', #128446 ) ;
#76433=AXIS2_PLACEMENT_3D ( 'NONE', #44212, #22668, #112962 ) ;
#76434=DIRECTION ( 'NONE',  ( 0.000000000000000000, 0.000000000000000000, -1.000000000000000000 ) ) ;
#76435=DIRECTION ( 'NONE',  ( -0.000000000000000000, -1.000000000000000000, -0.000000000000000000 ) ) ;
#76436=CARTESIAN_POINT ( 'NONE',  ( -13.94999999999998685, 12.50000000000000000, 1.883746621131362931 ) ) ;
#76437=AXIS2_PLACEMENT_3D ( 'NONE', #60422, #19838, #50567 ) ;
#76438=EDGE_LOOP ( 'NONE', ( #118272, #57324 ) ) ;
#76439=CIRCLE ( 'NONE', #5315, 0.06509327318403745899 ) ;
#76440=EDGE_CURVE ( 'NONE', #7017, #29011, #110870, .T. ) ;
#76441=FACE_OUTER_BOUND ( 'NONE', #14335, .T. ) ;
#76442=AXIS2_PLACEMENT_3D ( 'NONE', #124392, #73335, #24893 ) ;
#76443=ORIENTED_EDGE ( 'NONE', *, *, #66827, .T. ) ;
#76444=CARTESIAN_POINT ( 'NONE',  ( 34.93074629423288258, -2.900242961789775809, -4.640733549233234001 ) ) ;
#76445=CARTESIAN_POINT ( 'NONE',  ( -5.850000000000021849, 2.500000000000000000, -1.472243186433550122 ) ) ;
#76446=CARTESIAN_POINT ( 'NONE',  ( -3.950000000000026379, 2.500000000000000000, 2.511473670974873507 ) ) ;
#76447=CARTESIAN_POINT ( 'NONE',  ( 17.88933034088942975, -0.4802206367769106254, 4.999988745079923191 ) ) ;
#76448=EDGE_CURVE ( 'NONE', #55993, #90336, #62785, .T. ) ;
#76449=ORIENTED_EDGE ( 'NONE', *, *, #11879, .F. ) ;
#76450=VERTEX_POINT ( 'NONE', #70154 ) ;
#76451=ORIENTED_EDGE ( 'NONE', *, *, #112665, .T. ) ;
#76452=CARTESIAN_POINT ( 'NONE',  ( 10.19999999999991047, 2.500000000000000000, -3.883716857408426648 ) ) ;
#76453=DIRECTION ( 'NONE',  ( 0.000000000000000000, 1.000000000000000000, 0.000000000000000000 ) ) ;
#76454=EDGE_CURVE ( 'NONE', #114720, #55263, #35681, .T. ) ;
#76455=ADVANCED_FACE ( 'NONE', ( #60961 ), #78697, .T. ) ;
#76456=CARTESIAN_POINT ( 'NONE',  ( -6.250000000000015987, 12.50000000000000000, 1.407149913249508000 ) ) ;
#76457=EDGE_CURVE ( 'NONE', #108866, #6668, #9292, .T. ) ;
#76458=FACE_BOUND ( 'NONE', #41573, .T. ) ;
#76459=EDGE_CURVE ( 'NONE', #58766, #17273, #22352, .T. ) ;
#76460=DIRECTION ( 'NONE',  ( 0.000000000000000000, 1.000000000000000000, 0.000000000000000000 ) ) ;
#76461=CIRCLE ( 'NONE', #63849, 0.06509327318403745899 ) ;
#76462=DIRECTION ( 'NONE',  ( -0.000000000000000000, -1.000000000000000000, -0.000000000000000000 ) ) ;
#76463=DIRECTION ( 'NONE',  ( 0.000000000000000000, 1.000000000000000000, 0.000000000000000000 ) ) ;
#76466=EDGE_CURVE ( 'NONE', #66361, #74337, #13134, .T. ) ;
#76468=AXIS2_PLACEMENT_3D ( 'NONE', #79876, #72647, #101454 ) ;
#76469=CARTESIAN_POINT ( 'NONE',  ( -2.100000000000033396, 2.500000000000000000, -5.122947341949753763 ) ) ;
#76470=EDGE_CURVE ( 'NONE', #66532, #62883, #31474, .T. ) ;
#76471=FACE_OUTER_BOUND ( 'NONE', #27694, .T. ) ;
#76472=CONICAL_SURFACE ( 'NONE', #128818, 0.1000000000000000056, 0.003490658503988666988 ) ;
#76473=EDGE_CURVE ( 'NONE', #46102, #86677, #96200, .T. ) ;
#76474=EDGE_CURVE ( 'NONE', #54885, #119497, #20997, .T. ) ;
#76475=DIRECTION ( 'NONE',  ( 0.000000000000000000, -0.9999939076577903929, 0.003490651415223739937 ) ) ;
#76476=AXIS2_PLACEMENT_3D ( 'NONE', #37360, #76633, #67415 ) ;
#76477=VERTEX_POINT ( 'NONE', #73355 ) ;
#76478=EDGE_LOOP ( 'NONE', ( #123666, #40745 ) ) ;
#76479=VERTEX_POINT ( 'NONE', #3970 ) ;
#76480=ORIENTED_EDGE ( 'NONE', *, *, #13295, .F. ) ;
#76481=CARTESIAN_POINT ( 'NONE',  ( 2.899999999999943956, 2.500000000000000000, 4.330127018922196314 ) ) ;
#76482=FACE_BOUND ( 'NONE', #124058, .T. ) ;
#76483=ADVANCED_FACE ( 'NONE', ( #11856 ), #100423, .T. ) ;
#76484=FACE_OUTER_BOUND ( 'NONE', #46526, .T. ) ;
#76485=CIRCLE ( 'NONE', #51361, 0.1000000000000002554 ) ;
#76486=DIRECTION ( 'NONE',  ( 0.000000000000000000, 0.000000000000000000, 1.000000000000000000 ) ) ;
#76487=AXIS2_PLACEMENT_3D ( 'NONE', #108708, #118523, #88411 ) ;
#76488=AXIS2_PLACEMENT_3D ( 'NONE', #104187, #11931, #63628 ) ;
#76489=VERTEX_POINT ( 'NONE', #52431 ) ;
#76490=FACE_OUTER_BOUND ( 'NONE', #114361, .T. ) ;
#76491=DIRECTION ( 'NONE',  ( -0.000000000000000000, 1.000000000000000000, -0.000000000000000000 ) ) ;
#76492=ORIENTED_EDGE ( 'NONE', *, *, #119742, .T. ) ;
#76493=CARTESIAN_POINT ( 'NONE',  ( 105.5000000000000142, 0.000000000000000000, 0.000000000000000000 ) ) ;
#76494=DIRECTION ( 'NONE',  ( 0.000000000000000000, 0.000000000000000000, 1.000000000000000000 ) ) ;
#76495=VECTOR ( 'NONE', #66320, 1000.000000000000000 ) ;
#76496=CONICAL_SURFACE ( 'NONE', #97410, 0.1000000000000000472, 0.003490658503988666988 ) ;
#76497=ORIENTED_EDGE ( 'NONE', *, *, #52122, .T. ) ;
#76498=LINE ( 'NONE', #96756, #111333 ) ;
#76499=CARTESIAN_POINT ( 'NONE',  ( -12.49999999999999289, 2.500000000000000000, 4.922947341949748257 ) ) ;
#76500=ORIENTED_EDGE ( 'NONE', *, *, #37788, .F. ) ;
#76501=CARTESIAN_POINT ( 'NONE',  ( -1.650000000000035216, 2.500000000000000000, -1.472243186433550122 ) ) ;
#76502=DIRECTION ( 'NONE',  ( 0.000000000000000000, 1.000000000000000000, 0.000000000000000000 ) ) ;
#76503=VERTEX_POINT ( 'NONE', #32178 ) ;
#76504=DIRECTION ( 'NONE',  ( 0.000000000000000000, 0.000000000000000000, -1.000000000000000000 ) ) ;
#76505=EDGE_LOOP ( 'NONE', ( #19554, #5018 ) ) ;
#76506=ORIENTED_EDGE ( 'NONE', *, *, #84429, .T. ) ;
#76507=FACE_OUTER_BOUND ( 'NONE', #82488, .T. ) ;
#76508=VERTEX_POINT ( 'NONE', #94282 ) ;
#76509=DIRECTION ( 'NONE',  ( 0.000000000000000000, -0.9999939076577903929, 0.003490651415223739937 ) ) ;
#76510=CARTESIAN_POINT ( 'NONE',  ( 4.999999999999971578, 2.500000000000000000, -2.276824562219559311E-15 ) ) ;
#76511=EDGE_CURVE ( 'NONE', #11005, #102405, #41351, .T. ) ;
#76512=AXIS2_PLACEMENT_3D ( 'NONE', #4676, #85196, #26291 ) ;
#76513=VERTEX_POINT ( 'NONE', #23619 ) ;
#76514=AXIS2_PLACEMENT_3D ( 'NONE', #47930, #77380, #9282 ) ;
#76515=CARTESIAN_POINT ( 'NONE',  ( -1.650000000000034772, 2.500000000000000000, 5.702370205355745014 ) ) ;
#76516=EDGE_CURVE ( 'NONE', #55744, #87232, #89949, .T. ) ;
#76517=CARTESIAN_POINT ( 'NONE',  ( -4.350000000000023626, 12.50000000000000000, 6.841600689897072485 ) ) ;
#76518=DIRECTION ( 'NONE',  ( 0.000000000000000000, 0.000000000000000000, 1.000000000000000000 ) ) ;
#76519=CARTESIAN_POINT ( 'NONE',  ( -5.600000000000023626, 12.50000000000000000, -3.983716857408426293 ) ) ;
#76520=CARTESIAN_POINT ( 'NONE',  ( 11.89999999999990443, 12.50000000000000000, 0.3464101615137736845 ) ) ;
#76521=CARTESIAN_POINT ( 'NONE',  ( 7.699999999999923794, 12.50000000000000000, 4.741630453620009789 ) ) ;
#76523=VECTOR ( 'NONE', #31880, 1000.000000000000000 ) ;
#76524=VERTEX_POINT ( 'NONE', #3338 ) ;
#76525=VERTEX_POINT ( 'NONE', #104118 ) ;
#76526=CARTESIAN_POINT ( 'NONE',  ( -7.500000000000015099, 2.500000000000000000, -0.6928203230275541413 ) ) ;
#76527=FACE_OUTER_BOUND ( 'NONE', #117828, .T. ) ;
#76528=CARTESIAN_POINT ( 'NONE',  ( 5.399999999999934630, 2.500000000000000000, 0.6928203230275494784 ) ) ;
#76529=ORIENTED_EDGE ( 'NONE', *, *, #85061, .F. ) ;
#76531=VERTEX_POINT ( 'NONE', #121176 ) ;
#76532=CARTESIAN_POINT ( 'NONE',  ( -6.900000000000019007, 2.500000000000000000, -0.3464101615137783474 ) ) ;
#76533=CIRCLE ( 'NONE', #89136, 0.1000000000000002554 ) ;
#76534=LINE ( 'NONE', #85693, #119609 ) ;
#76535=FACE_OUTER_BOUND ( 'NONE', #114577, .T. ) ;
#76536=CIRCLE ( 'NONE', #15879, 0.06509327318403745899 ) ;
#76538=DIRECTION ( 'NONE',  ( -0.000000000000000000, 1.000000000000000000, -0.000000000000000000 ) ) ;
#76540=DIRECTION ( 'NONE',  ( 0.000000000000000000, 0.000000000000000000, -1.000000000000000000 ) ) ;
#76541=DIRECTION ( 'NONE',  ( 0.000000000000000000, 0.000000000000000000, 1.000000000000000000 ) ) ;
#76542=LINE ( 'NONE', #106633, #44664 ) ;
#76544=EDGE_LOOP ( 'NONE', ( #37100, #22827 ) ) ;
#76545=PLANE ( 'NONE',  #54999 ) ;
#76547=ORIENTED_EDGE ( 'NONE', *, *, #112115, .T. ) ;
#76548=DIRECTION ( 'NONE',  ( 0.000000000000000000, 0.000000000000000000, 1.000000000000000000 ) ) ;
#76549=CARTESIAN_POINT ( 'NONE',  ( -1.450000000000036371, 2.500000000000000000, 2.611473670974873151 ) ) ;
#76550=DIRECTION ( 'NONE',  ( 0.000000000000000000, -0.9999939076577903929, 0.003490651415223739937 ) ) ;
#76551=CARTESIAN_POINT ( 'NONE',  ( -9.400000000000009237, 2.500000000000000000, -4.776537180435973973 ) ) ;
#76552=DIRECTION ( 'NONE',  ( 0.000000000000000000, 1.000000000000000000, 0.000000000000000000 ) ) ;
#76553=PLANE ( 'NONE',  #15662 ) ;
#76554=CIRCLE ( 'NONE', #95617, 0.1000000000000002554 ) ;
#76555=DIRECTION ( 'NONE',  ( 0.000000000000000000, -0.9999939076577903929, 0.003490651415223739937 ) ) ;
#76556=VERTEX_POINT ( 'NONE', #63553 ) ;
#76557=DIRECTION ( 'NONE',  ( -0.000000000000000000, 1.000000000000000000, -0.000000000000000000 ) ) ;
#76558=CONICAL_SURFACE ( 'NONE', #30603, 0.1000000000000002554, 0.003490658503988666988 ) ;
#76559=CIRCLE ( 'NONE', #68228, 0.1000000000000002554 ) ;
#76560=AXIS2_PLACEMENT_3D ( 'NONE', #122525, #62325, #121872 ) ;
#76562=ORIENTED_EDGE ( 'NONE', *, *, #106310, .F. ) ;
#76563=ORIENTED_EDGE ( 'NONE', *, *, #124276, .T. ) ;
#76564=CIRCLE ( 'NONE', #86920, 0.09999999999999982514 ) ;
#76565=ORIENTED_EDGE ( 'NONE', *, *, #33479, .T. ) ;
#76566=ADVANCED_FACE ( 'NONE', ( #121814 ), #50257, .T. ) ;
#76567=VERTEX_POINT ( 'NONE', #103472 ) ;
#76568=EDGE_CURVE ( 'NONE', #109647, #34236, #69113, .T. ) ;
#76569=ORIENTED_EDGE ( 'NONE', *, *, #69574, .F. ) ;
#76570=DIRECTION ( 'NONE',  ( 0.000000000000000000, 0.000000000000000000, 1.000000000000000000 ) ) ;
#76571=PLANE ( 'NONE',  #39447 ) ;
#76572=VECTOR ( 'NONE', #97378, 1000.000000000000000 ) ;
#76573=EDGE_LOOP ( 'NONE', ( #91359, #20240 ) ) ;
#76574=DIRECTION ( 'NONE',  ( 0.000000000000000000, 0.000000000000000000, 1.000000000000000000 ) ) ;
#76575=LINE ( 'NONE', #116481, #80077 ) ;
#76576=VECTOR ( 'NONE', #28070, 1000.000000000000000 ) ;
#76577=AXIS2_PLACEMENT_3D ( 'NONE', #11122, #82474, #62191 ) ;
#76578=DIRECTION ( 'NONE',  ( 0.000000000000000000, 0.000000000000000000, 1.000000000000000000 ) ) ;
#76579=ORIENTED_EDGE ( 'NONE', *, *, #94154, .T. ) ;
#76580=ADVANCED_FACE ( 'NONE', ( #72725 ), #33541, .T. ) ;
#76581=CARTESIAN_POINT ( 'NONE',  ( -5.650000000000023448, 2.500000000000000000, -2.511473670974877948 ) ) ;
#76582=LINE ( 'NONE', #5248, #12184 ) ;
#76583=ORIENTED_EDGE ( 'NONE', *, *, #74021, .T. ) ;
#76584=VERTEX_POINT ( 'NONE', #82557 ) ;
#76585=ORIENTED_EDGE ( 'NONE', *, *, #10557, .F. ) ;
#76586=CARTESIAN_POINT ( 'NONE',  ( -2.500000000000031086, 2.500000000000000000, 3.637306695894644726 ) ) ;
#76588=EDGE_CURVE ( 'NONE', #13198, #122791, #112650, .T. ) ;
#76589=EDGE_LOOP ( 'NONE', ( #43655, #66577 ) ) ;
#76590=CARTESIAN_POINT ( 'NONE',  ( 1.649999999999949729, 2.500000000000000000, 5.802370205355744659 ) ) ;
#76591=CARTESIAN_POINT ( 'NONE',  ( -9.150000000000009237, 12.50000000000000000, -2.230156782645139391 ) ) ;
#76592=DIRECTION ( 'NONE',  ( 0.000000000000000000, 0.000000000000000000, -1.000000000000000000 ) ) ;
#76593=CARTESIAN_POINT ( 'NONE',  ( -7.500000000000011546, 2.500000000000000000, 3.537306695894645081 ) ) ;
#76594=EDGE_CURVE ( 'NONE', #25630, #117051, #102806, .T. ) ;
#76595=VERTEX_POINT ( 'NONE', #115860 ) ;
#76596=AXIS2_PLACEMENT_3D ( 'NONE', #9865, #89709, #110004 ) ;
#76597=CARTESIAN_POINT ( 'NONE',  ( 5.399999999999933742, 12.50000000000000000, -2.385244779468109755E-15 ) ) ;
#76598=CIRCLE ( 'NONE', #114249, 0.06509327318403745899 ) ;
#76599=ORIENTED_EDGE ( 'NONE', *, *, #58854, .F. ) ;
#76600=ORIENTED_EDGE ( 'NONE', *, *, #115422, .F. ) ;
#76601=EDGE_CURVE ( 'NONE', #60131, #66442, #39806, .T. ) ;
#76602=EDGE_LOOP ( 'NONE', ( #51892, #13007 ) ) ;
#76603=EDGE_CURVE ( 'NONE', #61095, #110247, #44002, .T. ) ;
#76604=DIRECTION ( 'NONE',  ( -0.000000000000000000, 1.000000000000000000, -0.000000000000000000 ) ) ;
#76605=ADVANCED_FACE ( 'NONE', ( #27462 ), #4254, .T. ) ;
#76606=FACE_BOUND ( 'NONE', #115702, .T. ) ;
#76607=EDGE_CURVE ( 'NONE', #85332, #110789, #16973, .T. ) ;
#76608=DIRECTION ( 'NONE',  ( 0.000000000000000000, -0.9999939076577903929, 0.003490651415223739937 ) ) ;
#76609=DIRECTION ( 'NONE',  ( -0.000000000000000000, -1.000000000000000000, -0.000000000000000000 ) ) ;
#76610=CONICAL_SURFACE ( 'NONE', #103798, 0.1000000000000002554, 0.003490658503988666988 ) ;
#76611=CONICAL_SURFACE ( 'NONE', #82882, 0.1000000000000000472, 0.003490658503988666988 ) ;
#76612=CARTESIAN_POINT ( 'NONE',  ( 10.79999999999991012, 12.50000000000000000, 4.265033745738159077 ) ) ;
#76613=EDGE_CURVE ( 'NONE', #98705, #57456, #18929, .T. ) ;
#76614=VERTEX_POINT ( 'NONE', #16348 ) ;
#76615=CARTESIAN_POINT ( 'NONE',  ( -11.44999999999999751, 2.500000000000000000, -6.841600689897074261 ) ) ;
#76616=CARTESIAN_POINT ( 'NONE',  ( -5.800000000000018474, 2.500000000000000000, 0.09999999999999772959 ) ) ;
#76617=EDGE_CURVE ( 'NONE', #81382, #41325, #36021, .T. ) ;
#76618=CARTESIAN_POINT ( 'NONE',  ( 15.83209681635554666, 2.500000000000000000, 5.404881881984142211 ) ) ;
#76619=DIRECTION ( 'NONE',  ( 0.000000000000000000, 1.000000000000000000, 0.000000000000000000 ) ) ;
#76620=ORIENTED_EDGE ( 'NONE', *, *, #105278, .T. ) ;
#76621=CONICAL_SURFACE ( 'NONE', #20186, 0.09999999999999982514, 0.003490658503988666988 ) ;
#76622=CONICAL_SURFACE ( 'NONE', #9723, 0.1000000000000002554, 0.003490658503988666988 ) ;
#76623=CARTESIAN_POINT ( 'NONE',  ( -8.550000000000011369, 12.50000000000000000, -2.511473670974877948 ) ) ;
#76624=CONICAL_SURFACE ( 'NONE', #97540, 0.1000000000000000472, 0.003490658503988666988 ) ;
#76626=DIRECTION ( 'NONE',  ( 0.000000000000000000, 0.000000000000000000, 1.000000000000000000 ) ) ;
#76627=ORIENTED_EDGE ( 'NONE', *, *, #30411, .F. ) ;
#76628=CARTESIAN_POINT ( 'NONE',  ( 11.24999999999994493, 12.50000000000000000, 6.495190528383297135 ) ) ;
#76629=ADVANCED_FACE ( 'NONE', ( #65466 ), #96207, .T. ) ;
#76630=DIRECTION ( 'NONE',  ( -0.000000000000000000, -1.000000000000000000, -0.000000000000000000 ) ) ;
#76631=FACE_BOUND ( 'NONE', #5780, .T. ) ;
#76632=EDGE_CURVE ( 'NONE', #1197, #38017, #77432, .T. ) ;
#76633=DIRECTION ( 'NONE',  ( 0.000000000000000000, 1.000000000000000000, 0.000000000000000000 ) ) ;
#76634=ORIENTED_EDGE ( 'NONE', *, *, #53878, .T. ) ;
#76635=FACE_OUTER_BOUND ( 'NONE', #6427, .T. ) ;
#76636=VERTEX_POINT ( 'NONE', #66753 ) ;
#76639=AXIS2_PLACEMENT_3D ( 'NONE', #81013, #112411, #41108 ) ;
#76640=EDGE_LOOP ( 'NONE', ( #125012, #27346, #89508, #87374 ) ) ;
#76642=AXIS2_PLACEMENT_3D ( 'NONE', #29028, #10017, #88569 ) ;
#76643=PLANE ( 'NONE',  #59512 ) ;
#76644=AXIS2_PLACEMENT_3D ( 'NONE', #125386, #46836, #64521 ) ;
#76645=CARTESIAN_POINT ( 'NONE',  ( -7.300000000000014921, 12.50000000000000000, 4.676537180435972552 ) ) ;
#76646=CARTESIAN_POINT ( 'NONE',  ( -4.600000000000028066, 12.50000000000000000, -3.637306695894650055 ) ) ;
#76647=AXIS2_PLACEMENT_3D ( 'NONE', #79696, #29972, #69888 ) ;
#76648=VERTEX_POINT ( 'NONE', #55005 ) ;
#76649=AXIS2_PLACEMENT_3D ( 'NONE', #25420, #55553, #54891 ) ;
#76650=FACE_OUTER_BOUND ( 'NONE', #67871, .T. ) ;
#76651=DIRECTION ( 'NONE',  ( 0.000000000000000000, 0.000000000000000000, 1.000000000000000000 ) ) ;
#76652=DIRECTION ( 'NONE',  ( 0.000000000000000000, 0.000000000000000000, -1.000000000000000000 ) ) ;
#76653=CARTESIAN_POINT ( 'NONE',  ( 18.46077503350462479, 0.2574728941691944994, -4.048716373199866325 ) ) ;
#76654=VERTEX_POINT ( 'NONE', #125667 ) ;
#76655=DIRECTION ( 'NONE',  ( 0.000000000000000000, 1.000000000000000000, 0.000000000000000000 ) ) ;
#76656=VERTEX_POINT ( 'NONE', #37323 ) ;
#76657=AXIS2_PLACEMENT_3D ( 'NONE', #98237, #39356, #108706 ) ;
#76658=CARTESIAN_POINT ( 'NONE',  ( 0.4499999999999552136, 12.50000000000000000, 6.430097255199259010 ) ) ;
#76659=DIRECTION ( 'NONE',  ( 0.000000000000000000, 0.000000000000000000, 1.000000000000000000 ) ) ;
#76660=CIRCLE ( 'NONE', #118418, 0.06509327318403743123 ) ;
#76662=CARTESIAN_POINT ( 'NONE',  ( -4.150000000000025224, 2.500000000000000000, 2.857883832488649301 ) ) ;
#76663=CARTESIAN_POINT ( 'NONE',  ( 17.50000000000000000, -2.499999999999999556, -3.333333333333330373 ) ) ;
#76664=ADVANCED_FACE ( 'NONE', ( #25532 ), #94946, .T. ) ;
#76665=CARTESIAN_POINT ( 'NONE',  ( -5.650000000000019895, 2.500000000000000000, 1.918653347947321564 ) ) ;
#76666=CIRCLE ( 'NONE', #9764, 0.1000000000000002554 ) ;
#76667=AXIS2_PLACEMENT_3D ( 'NONE', #114488, #54919, #85025 ) ;
#76668=LINE ( 'NONE', #16421, #69562 ) ;
#76670=DIRECTION ( 'NONE',  ( 0.000000000000000000, 1.000000000000000000, 0.000000000000000000 ) ) ;
#76671=EDGE_CURVE ( 'NONE', #20888, #80635, #117123, .T. ) ;
#76672=CARTESIAN_POINT ( 'NONE',  ( 10.39999999999990976, 12.50000000000000000, 4.265033745738159077 ) ) ;
#76673=CARTESIAN_POINT ( 'NONE',  ( -4.150000000000024336, 12.50000000000000000, 2.165063509461097713 ) ) ;
#76674=DIRECTION ( 'NONE',  ( 0.000000000000000000, -0.000000000000000000, 1.000000000000000000 ) ) ;
#76675=LINE ( 'NONE', #28218, #9700 ) ;
#76676=ORIENTED_EDGE ( 'NONE', *, *, #116326, .T. ) ;
#76677=ORIENTED_EDGE ( 'NONE', *, *, #55470, .F. ) ;
#76678=CARTESIAN_POINT ( 'NONE',  ( -11.24999999999996447, 12.50000000000000000, -2.165063509461097713 ) ) ;
#76679=ORIENTED_EDGE ( 'NONE', *, *, #8376, .T. ) ;
#76680=DIRECTION ( 'NONE',  ( -0.000000000000000000, 1.000000000000000000, -0.000000000000000000 ) ) ;
#76681=VERTEX_POINT ( 'NONE', #7184 ) ;
#76683=ORIENTED_EDGE ( 'NONE', *, *, #1078, .T. ) ;
#76684=AXIS2_PLACEMENT_3D ( 'NONE', #107744, #18061, #58011 ) ;
#76685=DIRECTION ( 'NONE',  ( 0.000000000000000000, 0.000000000000000000, 1.000000000000000000 ) ) ;
#76686=CARTESIAN_POINT ( 'NONE',  ( -11.44999999999999751, 12.50000000000000000, 6.148780366869520897 ) ) ;
#76687=DIRECTION ( 'NONE',  ( 0.000000000000000000, -0.000000000000000000, 1.000000000000000000 ) ) ;
#76688=CARTESIAN_POINT ( 'NONE',  ( -5.450000000000023270, 12.50000000000000000, -6.560283801567339701 ) ) ;
#76689=DIRECTION ( 'NONE',  ( 0.000000000000000000, 0.000000000000000000, 1.000000000000000000 ) ) ;
#76690=CARTESIAN_POINT ( 'NONE',  ( 0.1999999999999567124, 12.50000000000000000, -3.983716857408426293 ) ) ;
#76691=ORIENTED_EDGE ( 'NONE', *, *, #82868, .F. ) ;
#76692=DIRECTION ( 'NONE',  ( 0.000000000000000000, 0.000000000000000000, 1.000000000000000000 ) ) ;
#76693=VERTEX_POINT ( 'NONE', #77229 ) ;
#76694=CONICAL_SURFACE ( 'NONE', #120608, 0.09999999999999982514, 0.003490658503988666988 ) ;
#76695=ORIENTED_EDGE ( 'NONE', *, *, #25304, .T. ) ;
#76696=ORIENTED_EDGE ( 'NONE', *, *, #43569, .T. ) ;
#76697=ORIENTED_EDGE ( 'NONE', *, *, #105553, .F. ) ;
#76698=VECTOR ( 'NONE', #46808, 1000.000000000000000 ) ;
#76699=CARTESIAN_POINT ( 'NONE',  ( -10.60000000000000142, 12.50000000000000000, -0.2813168883297408329 ) ) ;
#76700=EDGE_LOOP ( 'NONE', ( #127205, #81673, #95908, #114679 ) ) ;
#76701=ORIENTED_EDGE ( 'NONE', *, *, #39922, .F. ) ;
#76702=CIRCLE ( 'NONE', #36996, 0.06509327318403745899 ) ;
#76703=ADVANCED_FACE ( 'NONE', ( #47137 ), #87040, .T. ) ;
#76704=CARTESIAN_POINT ( 'NONE',  ( -10.40000000000000213, 12.50000000000000000, 0.7579135962115869374 ) ) ;
#76705=CARTESIAN_POINT ( 'NONE',  ( 6.649999999999928413, 2.500000000000000000, 1.472243186433545459 ) ) ;
#76706=CARTESIAN_POINT ( 'NONE',  ( 10.44999999999991047, 2.500000000000000000, 2.265063509461097357 ) ) ;
#76707=CARTESIAN_POINT ( 'NONE',  ( 11.64999999999990798, 2.500000000000000000, 5.802370205355744659 ) ) ;
#76708=DIRECTION ( 'NONE',  ( -0.000000000000000000, 1.000000000000000000, -0.000000000000000000 ) ) ;
#76709=ORIENTED_EDGE ( 'NONE', *, *, #34854, .T. ) ;
#76710=DIRECTION ( 'NONE',  ( 0.000000000000000000, 0.000000000000000000, 1.000000000000000000 ) ) ;
#76711=CIRCLE ( 'NONE', #101845, 0.09999999999999982514 ) ;
#76712=ADVANCED_FACE ( 'NONE', ( #44551 ), #74648, .T. ) ;
#76713=EDGE_LOOP ( 'NONE', ( #57431, #88975, #100138, #48860 ) ) ;
#76714=DIRECTION ( 'NONE',  ( -0.000000000000000000, 1.000000000000000000, -0.000000000000000000 ) ) ;
#76715=AXIS2_PLACEMENT_3D ( 'NONE', #83417, #25768, #63114 ) ;
#76716=EDGE_LOOP ( 'NONE', ( #71368, #15567 ) ) ;
#76717=DIRECTION ( 'NONE',  ( -0.000000000000000000, 1.000000000000000000, -0.000000000000000000 ) ) ;
#76718=EDGE_LOOP ( 'NONE', ( #39616, #47697, #89717, #115155 ) ) ;
#76719=ADVANCED_FACE ( 'NONE', ( #5255 ), #14721, .T. ) ;
#76720=ADVANCED_FACE ( 'NONE', ( #75292 ), #16769, .T. ) ;
#76721=VERTEX_POINT ( 'NONE', #98791 ) ;
#76722=FACE_OUTER_BOUND ( 'NONE', #62329, .T. ) ;
#76723=DIRECTION ( 'NONE',  ( -0.000000000000000000, 1.000000000000000000, -0.000000000000000000 ) ) ;
#76724=CARTESIAN_POINT ( 'NONE',  ( 11.24999999999991118, 2.500000000000000000, -2.957883832488653830 ) ) ;
#76725=DIRECTION ( 'NONE',  ( 0.000000000000000000, 1.000000000000000000, 0.000000000000000000 ) ) ;
#76726=CARTESIAN_POINT ( 'NONE',  ( -13.34999999999999076, 2.500000000000000000, 2.957883832488652942 ) ) ;
#76727=ORIENTED_EDGE ( 'NONE', *, *, #31586, .T. ) ;
#76728=CARTESIAN_POINT ( 'NONE',  ( -13.09999999999999254, 12.50000000000000000, -3.983716857408423628 ) ) ;
#76729=CARTESIAN_POINT ( 'NONE',  ( 1.249999999999986899, 2.500000000000000000, 6.595190528383296780 ) ) ;
#76730=EDGE_CURVE ( 'NONE', #121037, #32550, #19604, .T. ) ;
#76731=CARTESIAN_POINT ( 'NONE',  ( -5.000000000000024869, 2.500000000000000000, -5.022947341949754119 ) ) ;
#76732=CIRCLE ( 'NONE', #101778, 0.06509327318403745899 ) ;
#76733=PLANE ( 'NONE',  #88944 ) ;
#76734=CONICAL_SURFACE ( 'NONE', #103924, 0.1000000000000002554, 0.003490658503988666988 ) ;
#76735=CONICAL_SURFACE ( 'NONE', #32939, 0.1000000000000000472, 0.003490658503988666988 ) ;
#76736=DIRECTION ( 'NONE',  ( -0.000000000000000000, 1.000000000000000000, -0.000000000000000000 ) ) ;
#76737=ORIENTED_EDGE ( 'NONE', *, *, #119651, .T. ) ;
#76738=CIRCLE ( 'NONE', #124760, 0.06509327318403745899 ) ;
#76739=ORIENTED_EDGE ( 'NONE', *, *, #122751, .F. ) ;
#76740=DIRECTION ( 'NONE',  ( 0.000000000000000000, -0.000000000000000000, 1.000000000000000000 ) ) ;
#76741=CIRCLE ( 'NONE', #24416, 0.1000000000000002554 ) ;
#76743=CIRCLE ( 'NONE', #116437, 0.06509327318403745899 ) ;
#76744=LINE ( 'NONE', #105563, #27796 ) ;
#76745=DIRECTION ( 'NONE',  ( -0.000000000000000000, -1.000000000000000000, -0.000000000000000000 ) ) ;
#76746=AXIS2_PLACEMENT_3D ( 'NONE', #121180, #100884, #120541 ) ;
#76747=VERTEX_POINT ( 'NONE', #8473 ) ;
#76749=CARTESIAN_POINT ( 'NONE',  ( 10.59999999999991260, 2.500000000000000000, 0.3464101615137735735 ) ) ;
#76750=CONICAL_SURFACE ( 'NONE', #72645, 0.1000000000000002554, 0.003490658503988666988 ) ;
#76751=DIRECTION ( 'NONE',  ( 0.000000000000000000, 0.000000000000000000, 1.000000000000000000 ) ) ;
#76752=DIRECTION ( 'NONE',  ( 0.000000000000000000, 1.000000000000000000, 0.000000000000000000 ) ) ;
#76753=LINE ( 'NONE', #95107, #28773 ) ;
#76754=ORIENTED_EDGE ( 'NONE', *, *, #20042, .T. ) ;
#76755=CONICAL_SURFACE ( 'NONE', #37053, 0.1000000000000000472, 0.003490658503988666988 ) ;
#76756=ADVANCED_FACE ( 'NONE', ( #40556 ), #125632, .T. ) ;
#76757=AXIS2_PLACEMENT_3D ( 'NONE', #6164, #35025, #4873 ) ;
#76758=AXIS2_PLACEMENT_3D ( 'NONE', #43684, #14179, #12882 ) ;
#76759=DIRECTION ( 'NONE',  ( 0.000000000000000000, 0.000000000000000000, -1.000000000000000000 ) ) ;
#76760=FACE_OUTER_BOUND ( 'NONE', #113083, .T. ) ;
#76761=ORIENTED_EDGE ( 'NONE', *, *, #101131, .F. ) ;
#76762=EDGE_CURVE ( 'NONE', #120592, #50078, #6390, .T. ) ;
#76764=CARTESIAN_POINT ( 'NONE',  ( 0.7999999999999548583, 2.500000000000000000, 4.330127018922196314 ) ) ;
#76765=ADVANCED_FACE ( 'NONE', ( #39275 ), #128939, .T. ) ;
#76766=FACE_OUTER_BOUND ( 'NONE', #107296, .T. ) ;
#76767=EDGE_LOOP ( 'NONE', ( #45575, #92284 ) ) ;
#76768=LINE ( 'NONE', #38128, #111664 ) ;
#76769=EDGE_CURVE ( 'NONE', #7349, #89205, #102557, .T. ) ;
#76770=ADVANCED_FACE ( 'NONE', ( #49726 ), #25275, .T. ) ;
#76771=EDGE_LOOP ( 'NONE', ( #114936, #61080, #77735, #6471 ) ) ;
#76772=DIRECTION ( 'NONE',  ( 0.000000000000000000, 1.000000000000000000, 0.000000000000000000 ) ) ;
#76773=DIRECTION ( 'NONE',  ( 0.000000000000000000, 0.000000000000000000, 1.000000000000000000 ) ) ;
#76774=EDGE_CURVE ( 'NONE', #116336, #16823, #31561, .T. ) ;
#76775=VECTOR ( 'NONE', #35917, 1000.000000000000000 ) ;
#76776=ADVANCED_FACE ( 'NONE', ( #79805 ), #46136, .T. ) ;
#76777=CARTESIAN_POINT ( 'NONE',  ( 1.849999999999948130, 12.50000000000000000, 6.083687093685482772 ) ) ;
#76778=EDGE_LOOP ( 'NONE', ( #20029, #29227 ) ) ;
#76779=CARTESIAN_POINT ( 'NONE',  ( -10.00000000000000355, 2.500000000000000000, -0.6928203230275541413 ) ) ;
#76780=EDGE_CURVE ( 'NONE', #34168, #121648, #75463, .T. ) ;
#76782=ORIENTED_EDGE ( 'NONE', *, *, #80139, .F. ) ;
#76783=VERTEX_POINT ( 'NONE', #70632 ) ;
#76784=EDGE_CURVE ( 'NONE', #65382, #59496, #23145, .T. ) ;
#76785=CARTESIAN_POINT ( 'NONE',  ( -9.150000000000009237, 12.50000000000000000, -1.472243186433550122 ) ) ;
#76786=AXIS2_PLACEMENT_3D ( 'NONE', #31301, #21457, #89554 ) ;
#76787=AXIS2_PLACEMENT_3D ( 'NONE', #121333, #123276, #31673 ) ;
#76788=VERTEX_POINT ( 'NONE', #69998 ) ;
#76790=CARTESIAN_POINT ( 'NONE',  ( -12.09999999999999609, 12.50000000000000000, 0.6928203230275535862 ) ) ;
#76791=EDGE_LOOP ( 'NONE', ( #16719, #17856 ) ) ;
#76792=ORIENTED_EDGE ( 'NONE', *, *, #32799, .T. ) ;
#76793=DIRECTION ( 'NONE',  ( -4.274815082592931898E-19, -0.9999939076577903929, -0.003490651415223739937 ) ) ;
#76794=DIRECTION ( 'NONE',  ( 0.000000000000000000, 1.000000000000000000, 0.000000000000000000 ) ) ;
#76795=EDGE_LOOP ( 'NONE', ( #122909, #37743 ) ) ;
#76796=AXIS2_PLACEMENT_3D ( 'NONE', #49571, #70481, #18795 ) ;
#76797=CIRCLE ( 'NONE', #116490, 0.06509327318403745899 ) ;
#76798=DIRECTION ( 'NONE',  ( 0.000000000000000000, 0.000000000000000000, 1.000000000000000000 ) ) ;
#76799=CARTESIAN_POINT ( 'NONE',  ( 12.89999999999990266, 12.50000000000000000, 5.022947341949748790 ) ) ;
#76800=AXIS2_PLACEMENT_3D ( 'NONE', #119193, #9241, #18410 ) ;
#76801=CARTESIAN_POINT ( 'NONE',  ( 16.80832070732106232, -1.716026667539209516, -5.822501722885366604 ) ) ;
#76802=DIRECTION ( 'NONE',  ( 0.000000000000000000, 0.000000000000000000, 1.000000000000000000 ) ) ;
#76803=FACE_OUTER_BOUND ( 'NONE', #117386, .T. ) ;
#76804=CARTESIAN_POINT ( 'NONE',  ( 87.50000000000001421, -3.975350567648449740, -6.360562287258772152 ) ) ;
#76805=AXIS2_PLACEMENT_3D ( 'NONE', #78856, #87984, #87345 ) ;
#76806=CIRCLE ( 'NONE', #89324, 0.06509327318403745899 ) ;
#76807=CIRCLE ( 'NONE', #91466, 0.09999999999999982514 ) ;
#76808=ORIENTED_EDGE ( 'NONE', *, *, #106634, .T. ) ;
#76809=VERTEX_POINT ( 'NONE', #68049 ) ;
#76810=VERTEX_POINT ( 'NONE', #109925 ) ;
#76811=EDGE_LOOP ( 'NONE', ( #84428, #94916 ) ) ;
#76812=CARTESIAN_POINT ( 'NONE',  ( -0.8500000000000382805, 12.50000000000000000, -7.188010851410854052 ) ) ;
#76813=DIRECTION ( 'NONE',  ( 0.000000000000000000, 1.000000000000000000, 0.000000000000000000 ) ) ;
#76814=DIRECTION ( 'NONE',  ( 0.000000000000000000, 1.000000000000000000, 0.000000000000000000 ) ) ;
#76815=EDGE_LOOP ( 'NONE', ( #37940, #6852 ) ) ;
#76816=FACE_BOUND ( 'NONE', #85957, .T. ) ;
#76817=CARTESIAN_POINT ( 'NONE',  ( 4.149999999999939959, 2.500000000000000000, -2.065063509461102065 ) ) ;
#76818=DIRECTION ( 'NONE',  ( 0.000000000000000000, 0.000000000000000000, 1.000000000000000000 ) ) ;
#76819=DIRECTION ( 'NONE',  ( 0.000000000000000000, 1.000000000000000000, 0.000000000000000000 ) ) ;
#76820=CONICAL_SURFACE ( 'NONE', #120722, 0.09999999999999999167, 0.003490658503988666988 ) ;
#76821=ADVANCED_FACE ( 'NONE', ( #20248 ), #33620, .T. ) ;
#76822=CARTESIAN_POINT ( 'NONE',  ( -9.600000000000008527, 2.500000000000000000, 4.230127018922196669 ) ) ;
#76823=CARTESIAN_POINT ( 'NONE',  ( -3.150000000000029665, 12.50000000000000000, 6.841600689897072485 ) ) ;
#76824=AXIS2_PLACEMENT_3D ( 'NONE', #129341, #39673, #107739 ) ;
#76825=CARTESIAN_POINT ( 'NONE',  ( 0.4499999999999552136, 2.500000000000000000, 6.595190528383296780 ) ) ;
#76826=CARTESIAN_POINT ( 'NONE',  ( 4.349999999999940137, 12.50000000000000000, -6.841600689897078702 ) ) ;
#76827=FACE_OUTER_BOUND ( 'NONE', #77545, .T. ) ;
#76828=CARTESIAN_POINT ( 'NONE',  ( -11.84999999999999787, 2.500000000000000000, -2.611473670974873595 ) ) ;
#76829=CIRCLE ( 'NONE', #5785, 0.09999999999999982514 ) ;
#76830=LINE ( 'NONE', #116733, #27234 ) ;
#76831=EDGE_CURVE ( 'NONE', #105454, #47303, #8549, .T. ) ;
#76832=ORIENTED_EDGE ( 'NONE', *, *, #125365, .T. ) ;
#76833=CIRCLE ( 'NONE', #81041, 0.06509327318403743123 ) ;
#76834=EDGE_LOOP ( 'NONE', ( #5156, #52423, #36392, #28026 ) ) ;
#76835=ORIENTED_EDGE ( 'NONE', *, *, #42018, .T. ) ;
#76836=ORIENTED_EDGE ( 'NONE', *, *, #38288, .F. ) ;
#76837=DIRECTION ( 'NONE',  ( 0.000000000000000000, -0.000000000000000000, 1.000000000000000000 ) ) ;
#76838=DIRECTION ( 'NONE',  ( -0.000000000000000000, 1.000000000000000000, -0.000000000000000000 ) ) ;
#76839=EDGE_LOOP ( 'NONE', ( #89035, #110130 ) ) ;
#76840=ORIENTED_EDGE ( 'NONE', *, *, #56398, .T. ) ;
#76841=CONICAL_SURFACE ( 'NONE', #51705, 0.1000000000000000472, 0.003490658503988666988 ) ;
#76842=EDGE_LOOP ( 'NONE', ( #7378, #6687 ) ) ;
#76843=DIRECTION ( 'NONE',  ( 0.000000000000000000, 0.000000000000000000, -1.000000000000000000 ) ) ;
#76844=AXIS2_PLACEMENT_3D ( 'NONE', #37700, #9527, #118829 ) ;
#76845=CIRCLE ( 'NONE', #104025, 0.09999999999999982514 ) ;
#76846=CIRCLE ( 'NONE', #41253, 0.1000000000000002554 ) ;
#76847=CARTESIAN_POINT ( 'NONE',  ( 3.709550432145070076, -2.499999999998979483, 9.999999999913205428 ) ) ;
#76848=CARTESIAN_POINT ( 'NONE',  ( -9.600000000000008527, 2.500000000000000000, -3.637306695894645614 ) ) ;
#76849=CARTESIAN_POINT ( 'NONE',  ( 5.199999999999935341, 2.500000000000000000, -0.3464101615137783474 ) ) ;
#76851=CIRCLE ( 'NONE', #45551, 0.06509327318403745899 ) ;
#76852=EDGE_LOOP ( 'NONE', ( #112181, #5747, #67823, #108447 ) ) ;
#76854=AXIS2_PLACEMENT_3D ( 'NONE', #28410, #98411, #8738 ) ;
#76855=CIRCLE ( 'NONE', #81064, 0.1000000000000002554 ) ;
#76856=VERTEX_POINT ( 'NONE', #589 ) ;
#76857=VERTEX_POINT ( 'NONE', #20891 ) ;
#76858=CARTESIAN_POINT ( 'NONE',  ( 8.549999999999918998, 2.500000000000000000, -1.818653347947326138 ) ) ;
#76859=ORIENTED_EDGE ( 'NONE', *, *, #54007, .F. ) ;
#76860=EDGE_LOOP ( 'NONE', ( #37094, #33859, #67030, #49410 ) ) ;
#76861=DIRECTION ( 'NONE',  ( 0.000000000000000000, -0.000000000000000000, 1.000000000000000000 ) ) ;
#76862=EDGE_CURVE ( 'NONE', #122612, #79666, #100506, .T. ) ;
#76863=DIRECTION ( 'NONE',  ( 0.000000000000000000, 0.000000000000000000, 1.000000000000000000 ) ) ;
#76864=DIRECTION ( 'NONE',  ( -0.000000000000000000, -1.000000000000000000, -0.000000000000000000 ) ) ;
#76865=DIRECTION ( 'NONE',  ( 0.000000000000000000, 0.000000000000000000, 1.000000000000000000 ) ) ;
#76866=DIRECTION ( 'NONE',  ( -0.000000000000000000, 1.000000000000000000, -0.000000000000000000 ) ) ;
#76867=AXIS2_PLACEMENT_3D ( 'NONE', #68595, #28041, #37849 ) ;
#76868=ORIENTED_EDGE ( 'NONE', *, *, #46519, .T. ) ;
#76869=DIRECTION ( 'NONE',  ( 0.000000000000000000, 0.000000000000000000, 1.000000000000000000 ) ) ;
#76872=DIRECTION ( 'NONE',  ( 0.000000000000000000, 0.000000000000000000, 1.000000000000000000 ) ) ;
#76873=ORIENTED_EDGE ( 'NONE', *, *, #1862, .T. ) ;
#76874=DIRECTION ( 'NONE',  ( 0.000000000000000000, 0.000000000000000000, 1.000000000000000000 ) ) ;
#76875=CARTESIAN_POINT ( 'NONE',  ( -8.750000000000008882, 2.500000000000000000, 1.372243186433545370 ) ) ;
#76876=VERTEX_POINT ( 'NONE', #108618 ) ;
#76877=CARTESIAN_POINT ( 'NONE',  ( 14.14999999999989733, 12.50000000000000000, 2.857883832488649301 ) ) ;
#76878=EDGE_CURVE ( 'NONE', #12513, #3855, #127698, .T. ) ;
#76879=DIRECTION ( 'NONE',  ( 0.000000000000000000, 0.000000000000000000, 1.000000000000000000 ) ) ;
#76880=EDGE_CURVE ( 'NONE', #128103, #53498, #44078, .T. ) ;
#76881=EDGE_LOOP ( 'NONE', ( #72433, #86687, #81658, #94302 ) ) ;
#76883=CARTESIAN_POINT ( 'NONE',  ( 11.24999999999994316, 2.500000000000000000, 2.065063509461097624 ) ) ;
#76884=ORIENTED_EDGE ( 'NONE', *, *, #21936, .F. ) ;
#76885=VERTEX_POINT ( 'NONE', #72578 ) ;
#76886=DIRECTION ( 'NONE',  ( 0.000000000000000000, 0.000000000000000000, -1.000000000000000000 ) ) ;
#76887=FACE_OUTER_BOUND ( 'NONE', #104819, .T. ) ;
#76888=EDGE_CURVE ( 'NONE', #110798, #9926, #106760, .T. ) ;
#76890=DIRECTION ( 'NONE',  ( -0.000000000000000000, -1.000000000000000000, -0.000000000000000000 ) ) ;
#76891=AXIS2_PLACEMENT_3D ( 'NONE', #118715, #123074, #52392 ) ;
#76892=VECTOR ( 'NONE', #21639, 1000.000000000000000 ) ;
#76893=DIRECTION ( 'NONE',  ( 0.000000000000000000, 1.000000000000000000, 0.000000000000000000 ) ) ;
#76895=ORIENTED_EDGE ( 'NONE', *, *, #50637, .F. ) ;
#76896=FACE_OUTER_BOUND ( 'NONE', #61046, .T. ) ;
#76897=CIRCLE ( 'NONE', #20465, 0.06509327318403745899 ) ;
#76898=ORIENTED_EDGE ( 'NONE', *, *, #46411, .F. ) ;
#76899=AXIS2_PLACEMENT_3D ( 'NONE', #63846, #54025, #44190 ) ;
#76900=CARTESIAN_POINT ( 'NONE',  ( 7.299999999999926104, 12.50000000000000000, -0.3464101615137782364 ) ) ;
#76902=DIRECTION ( 'NONE',  ( 0.000000000000000000, 0.000000000000000000, 1.000000000000000000 ) ) ;
#76903=DIRECTION ( 'NONE',  ( 0.000000000000000000, 1.000000000000000000, 0.000000000000000000 ) ) ;
#76904=DIRECTION ( 'NONE',  ( 0.000000000000000000, 0.000000000000000000, 1.000000000000000000 ) ) ;
#76905=ORIENTED_EDGE ( 'NONE', *, *, #127941, .F. ) ;
#76906=CIRCLE ( 'NONE', #3739, 0.06509327318403745899 ) ;
#76907=CARTESIAN_POINT ( 'NONE',  ( 1.049999999999954525, 12.50000000000000000, -2.446380397790840266 ) ) ;
#76908=CIRCLE ( 'NONE', #20486, 0.09999999999999982514 ) ;
#76909=CONICAL_SURFACE ( 'NONE', #72811, 0.09999999999999982514, 0.003490658503988666988 ) ;
#76910=EDGE_LOOP ( 'NONE', ( #104280, #72537, #83494, #71173 ) ) ;
#76911=AXIS2_PLACEMENT_3D ( 'NONE', #32765, #111271, #22297 ) ;
#76912=CARTESIAN_POINT ( 'NONE',  ( -9.150000000000005684, 2.500000000000000000, 5.802370205355744659 ) ) ;
#76913=VECTOR ( 'NONE', #15230, 1000.000000000000000 ) ;
#76914=ORIENTED_EDGE ( 'NONE', *, *, #25909, .F. ) ;
#76915=EDGE_LOOP ( 'NONE', ( #48763, #77786, #9790, #28407 ) ) ;
#76916=CARTESIAN_POINT ( 'NONE',  ( 21.34481565588190577, 0.7053969147712814136, -2.184679923000765189 ) ) ;
#76917=EDGE_CURVE ( 'NONE', #75562, #96223, #12666, .T. ) ;
#76918=ADVANCED_FACE ( 'NONE', ( #51014 ), #71260, .T. ) ;
#76919=AXIS2_PLACEMENT_3D ( 'NONE', #89216, #68275, #39503 ) ;
#76920=ORIENTED_EDGE ( 'NONE', *, *, #96847, .T. ) ;
#76921=FACE_OUTER_BOUND ( 'NONE', #85044, .T. ) ;
#76923=EDGE_CURVE ( 'NONE', #118375, #73740, #84826, .T. ) ;
#76924=CIRCLE ( 'NONE', #53942, 0.1000000000000002554 ) ;
#76925=EDGE_CURVE ( 'NONE', #117196, #17735, #123487, .T. ) ;
#76926=CARTESIAN_POINT ( 'NONE',  ( 1.849999999999951017, 12.50000000000000000, -6.148780366869526226 ) ) ;
#76927=ORIENTED_EDGE ( 'NONE', *, *, #53814, .T. ) ;
#76928=AXIS2_PLACEMENT_3D ( 'NONE', #35243, #84323, #123596 ) ;
#76929=FACE_BOUND ( 'NONE', #71653, .T. ) ;
#76930=EDGE_CURVE ( 'NONE', #51911, #16954, #83784, .T. ) ;
#76931=CARTESIAN_POINT ( 'NONE',  ( 7.049999999999928768, 2.500000000000000000, 6.395190528383296602 ) ) ;
#76932=EDGE_LOOP ( 'NONE', ( #116397, #86467, #40527, #82805 ) ) ;
#76933=DIRECTION ( 'NONE',  ( 0.000000000000000000, 0.000000000000000000, 1.000000000000000000 ) ) ;
#76934=VECTOR ( 'NONE', #31307, 1000.000000000000000 ) ;
#76935=FACE_OUTER_BOUND ( 'NONE', #23722, .T. ) ;
#76936=VERTEX_POINT ( 'NONE', #111857 ) ;
#76937=EDGE_CURVE ( 'NONE', #107629, #121502, #108903, .T. ) ;
#76938=AXIS2_PLACEMENT_3D ( 'NONE', #40510, #57046, #7952 ) ;
#76939=CIRCLE ( 'NONE', #3782, 0.1000000000000000472 ) ;
#76940=EDGE_CURVE ( 'NONE', #2654, #101787, #51655, .T. ) ;
#76941=VERTEX_POINT ( 'NONE', #33931 ) ;
#76942=ORIENTED_EDGE ( 'NONE', *, *, #26549, .T. ) ;
#76943=PLANE ( 'NONE',  #121517 ) ;
#76944=DIRECTION ( 'NONE',  ( -4.274815082592931898E-19, -0.9999939076577903929, -0.003490651415223739937 ) ) ;
#76945=( BOUNDED_CURVE ( )  B_SPLINE_CURVE ( 2, ( #39664, #27881, #49479 ),
 .UNSPECIFIED., .F., .F. ) 
 B_SPLINE_CURVE_WITH_KNOTS ( ( 3, 3 ),
 ( 0.0008083180696977302617, 0.0008883710667521953468 ),
 .UNSPECIFIED. ) 
 CURVE ( )  GEOMETRIC_REPRESENTATION_ITEM ( )  RATIONAL_B_SPLINE_CURVE ( ( 0.9944676636816576210, 0.9972072019273532373, 1.000000000000000000 ) ) 
 REPRESENTATION_ITEM ( '' )  );
#76946=LINE ( 'NONE', #19291, #83966 ) ;
#76947=FACE_BOUND ( 'NONE', #5896, .T. ) ;
#76948=ORIENTED_EDGE ( 'NONE', *, *, #112115, .F. ) ;
#76949=CARTESIAN_POINT ( 'NONE',  ( 1.849999999999950573, 12.50000000000000000, 2.511473670974873507 ) ) ;
#76950=PLANE ( 'NONE',  #116982 ) ;
#76951=DIRECTION ( 'NONE',  ( -0.000000000000000000, 1.000000000000000000, -0.000000000000000000 ) ) ;
#76952=DIRECTION ( 'NONE',  ( -0.000000000000000000, -1.000000000000000000, -0.000000000000000000 ) ) ;
#76953=FACE_OUTER_BOUND ( 'NONE', #50449, .T. ) ;
#76954=LINE ( 'NONE', #35741, #122358 ) ;
#76955=CARTESIAN_POINT ( 'NONE',  ( 9.399999999999915090, 12.50000000000000000, -3.918623584224389056 ) ) ;
#76956=ORIENTED_EDGE ( 'NONE', *, *, #125765, .F. ) ;
#76957=ORIENTED_EDGE ( 'NONE', *, *, #71993, .T. ) ;
#76958=EDGE_LOOP ( 'NONE', ( #107001, #33238, #89556, #68532 ) ) ;
#76959=AXIS2_PLACEMENT_3D ( 'NONE', #47214, #51089, #101465 ) ;
#76960=CIRCLE ( 'NONE', #91622, 0.1000000000000000472 ) ;
#76961=VERTEX_POINT ( 'NONE', #21535 ) ;
#76962=EDGE_LOOP ( 'NONE', ( #100300, #46988 ) ) ;
#76963=CARTESIAN_POINT ( 'NONE',  ( 0.5999999999999612310, 2.500000000000000000, -0.4464101615137760493 ) ) ;
#76964=AXIS2_PLACEMENT_3D ( 'NONE', #59457, #49628, #107235 ) ;
#76965=PLANE ( 'NONE',  #6955 ) ;
#76966=ORIENTED_EDGE ( 'NONE', *, *, #83456, .F. ) ;
#76967=FACE_BOUND ( 'NONE', #99618, .T. ) ;
#76968=DIRECTION ( 'NONE',  ( -0.000000000000000000, -1.000000000000000000, -0.000000000000000000 ) ) ;
#76969=CIRCLE ( 'NONE', #22612, 0.1000000000000002554 ) ;
#76970=AXIS2_PLACEMENT_3D ( 'NONE', #13572, #52233, #21476 ) ;
#76971=DIRECTION ( 'NONE',  ( -4.274815082592931898E-19, -0.9999939076577903929, -0.003490651415223739937 ) ) ;
#76972=DIRECTION ( 'NONE',  ( 0.000000000000000000, 0.000000000000000000, -1.000000000000000000 ) ) ;
#76973=DIRECTION ( 'NONE',  ( 0.000000000000000000, 1.000000000000000000, 0.000000000000000000 ) ) ;
#76974=DIRECTION ( 'NONE',  ( 0.000000000000000000, 1.000000000000000000, 0.000000000000000000 ) ) ;
#76975=ORIENTED_EDGE ( 'NONE', *, *, #89005, .F. ) ;
#76976=DIRECTION ( 'NONE',  ( -0.000000000000000000, 1.000000000000000000, -0.000000000000000000 ) ) ;
#76977=VERTEX_POINT ( 'NONE', #122961 ) ;
#76978=EDGE_CURVE ( 'NONE', #118395, #67119, #91563, .T. ) ;
#76979=AXIS2_PLACEMENT_3D ( 'NONE', #28802, #68708, #108633 ) ;
#76980=ORIENTED_EDGE ( 'NONE', *, *, #75394, .F. ) ;
#76981=ORIENTED_EDGE ( 'NONE', *, *, #58926, .T. ) ;
#76982=DIRECTION ( 'NONE',  ( -0.000000000000000000, 1.000000000000000000, -0.000000000000000000 ) ) ;
#76983=CARTESIAN_POINT ( 'NONE',  ( 13.12246079422102341, 2.499999999999999112, 7.156134183588167552 ) ) ;
#76984=DIRECTION ( 'NONE',  ( -0.000000000000000000, 1.000000000000000000, -0.000000000000000000 ) ) ;
#76985=ORIENTED_EDGE ( 'NONE', *, *, #62963, .F. ) ;
#76986=CARTESIAN_POINT ( 'NONE',  ( 16.56576425165006228, 2.499999999999999556, -6.084390597445810123 ) ) ;
#76987=CIRCLE ( 'NONE', #20559, 0.06509327318403745899 ) ;
#76989=CARTESIAN_POINT ( 'NONE',  ( 3.749999999999942268, 12.50000000000000000, -1.472243186433550122 ) ) ;
#76991=CARTESIAN_POINT ( 'NONE',  ( -4.600000000000024514, 12.50000000000000000, 4.957854068765711553 ) ) ;
#76992=CARTESIAN_POINT ( 'NONE',  ( 15.39999999999989022, 12.50000000000000000, 0.06509327318403504425 ) ) ;
#76993=CIRCLE ( 'NONE', #72793, 0.06509327318403745899 ) ;
#76994=FACE_OUTER_BOUND ( 'NONE', #27436, .T. ) ;
#76995=ORIENTED_EDGE ( 'NONE', *, *, #3542, .F. ) ;
#76996=DIRECTION ( 'NONE',  ( 0.000000000000000000, 0.000000000000000000, 1.000000000000000000 ) ) ;
#76997=CIRCLE ( 'NONE', #127188, 0.06509327318403745899 ) ;
#76998=VERTEX_POINT ( 'NONE', #81112 ) ;
#76999=ORIENTED_EDGE ( 'NONE', *, *, #45037, .T. ) ;
#77001=CARTESIAN_POINT ( 'NONE',  ( -7.100000000000017408, 2.500000000000000000, -5.022947341949754119 ) ) ;
#77002=CARTESIAN_POINT ( 'NONE',  ( 1.849999999999950573, 2.500000000000000000, 2.511473670974873507 ) ) ;
#77003=CARTESIAN_POINT ( 'NONE',  ( -4.150000000000024336, 2.500000000000000000, 1.372243186433545370 ) ) ;
#77004=ORIENTED_EDGE ( 'NONE', *, *, #35316, .F. ) ;
#77005=CONICAL_SURFACE ( 'NONE', #83279, 0.09999999999999982514, 0.003490658503988666988 ) ;
#77006=ORIENTED_EDGE ( 'NONE', *, *, #115091, .T. ) ;
#77007=CARTESIAN_POINT ( 'NONE',  ( 11.84999999999990372, 2.500000000000000000, -6.148780366869526226 ) ) ;
#77008=AXIS2_PLACEMENT_3D ( 'NONE', #112018, #21046, #72100 ) ;
#77009=DIRECTION ( 'NONE',  ( -0.000000000000000000, 1.000000000000000000, -0.000000000000000000 ) ) ;
#77010=DIRECTION ( 'NONE',  ( 0.000000000000000000, 1.000000000000000000, 0.000000000000000000 ) ) ;
#77011=ORIENTED_EDGE ( 'NONE', *, *, #9097, .F. ) ;
#77012=ORIENTED_EDGE ( 'NONE', *, *, #41648, .T. ) ;
#77013=LINE ( 'NONE', #37741, #6337 ) ;
#77014=AXIS2_PLACEMENT_3D ( 'NONE', #35457, #104806, #96930 ) ;
#77015=VERTEX_POINT ( 'NONE', #121022 ) ;
#77016=FACE_OUTER_BOUND ( 'NONE', #116434, .T. ) ;
#77017=EDGE_CURVE ( 'NONE', #104132, #73436, #4336, .T. ) ;
#77018=CARTESIAN_POINT ( 'NONE',  ( 3.349999999999943689, 12.50000000000000000, 1.472243186433545459 ) ) ;
#77019=ORIENTED_EDGE ( 'NONE', *, *, #67291, .F. ) ;
#77020=DIRECTION ( 'NONE',  ( -0.000000000000000000, 1.000000000000000000, -0.000000000000000000 ) ) ;
#77021=CARTESIAN_POINT ( 'NONE',  ( 11.84999999999990372, 12.50000000000000000, 2.511473670974873507 ) ) ;
#77022=LINE ( 'NONE', #17436, #115745 ) ;
#77023=CIRCLE ( 'NONE', #20592, 0.09999999999999982514 ) ;
#77024=EDGE_CURVE ( 'NONE', #38979, #26349, #104701, .T. ) ;
#77025=DIRECTION ( 'NONE',  ( -4.274815082592931898E-19, -0.9999939076577903929, -0.003490651415223739937 ) ) ;
#77026=EDGE_CURVE ( 'NONE', #39885, #127091, #21084, .T. ) ;
#77027=VERTEX_POINT ( 'NONE', #52929 ) ;
#77028=DIRECTION ( 'NONE',  ( 0.000000000000000000, 0.000000000000000000, -1.000000000000000000 ) ) ;
#77029=CONICAL_SURFACE ( 'NONE', #29019, 0.1000000000000000472, 0.003490658503988666988 ) ;
#77030=AXIS2_PLACEMENT_3D ( 'NONE', #65304, #67895, #45693 ) ;
#77031=DIRECTION ( 'NONE',  ( -0.000000000000000000, -1.000000000000000000, -0.000000000000000000 ) ) ;
#77032=ADVANCED_FACE ( 'NONE', ( #113788 ), #58756, .T. ) ;
#77033=VERTEX_POINT ( 'NONE', #13632 ) ;
#77034=EDGE_CURVE ( 'NONE', #62185, #15358, #121432, .T. ) ;
#77035=ORIENTED_EDGE ( 'NONE', *, *, #104223, .F. ) ;
#77036=EDGE_CURVE ( 'NONE', #128073, #78150, #32673, .T. ) ;
#77038=DIRECTION ( 'NONE',  ( 0.000000000000000000, 1.000000000000000000, 0.000000000000000000 ) ) ;
#77039=EDGE_CURVE ( 'NONE', #36055, #54722, #2294, .T. ) ;
#77040=DIRECTION ( 'NONE',  ( 0.000000000000000000, -0.000000000000000000, 1.000000000000000000 ) ) ;
#77041=EDGE_CURVE ( 'NONE', #29442, #67610, #52474, .T. ) ;
#77042=LINE ( 'NONE', #126134, #43876 ) ;
#77043=DIRECTION ( 'NONE',  ( -4.274815082592931898E-19, -0.9999939076577903929, -0.003490651415223739937 ) ) ;
#77044=DIRECTION ( 'NONE',  ( -0.000000000000000000, -1.000000000000000000, -0.000000000000000000 ) ) ;
#77045=FACE_OUTER_BOUND ( 'NONE', #25788, .T. ) ;
#77046=CARTESIAN_POINT ( 'NONE',  ( 8.549999999999920774, 2.500000000000000000, 6.148780366869520897 ) ) ;
#77047=DIRECTION ( 'NONE',  ( 0.000000000000000000, 0.000000000000000000, 1.000000000000000000 ) ) ;
#77048=AXIS2_PLACEMENT_3D ( 'NONE', #11259, #92397, #81304 ) ;
#77049=ADVANCED_FACE ( 'NONE', ( #126175 ), #123576, .T. ) ;
#77050=FACE_OUTER_BOUND ( 'NONE', #3143, .T. ) ;
#77051=CIRCLE ( 'NONE', #37352, 0.06509327318403745899 ) ;
#77052=VECTOR ( 'NONE', #110207, 1000.000000000000000 ) ;
#77054=CIRCLE ( 'NONE', #108433, 0.06509327318403745899 ) ;
#77055=DIRECTION ( 'NONE',  ( 0.000000000000000000, 0.000000000000000000, 1.000000000000000000 ) ) ;
#77056=CARTESIAN_POINT ( 'NONE',  ( 8.149999999999920419, 2.500000000000000000, -1.918653347947325782 ) ) ;
#77057=CARTESIAN_POINT ( 'NONE',  ( 2.049999999999950084, 2.500000000000000000, -2.265063509461101798 ) ) ;
#77058=CARTESIAN_POINT ( 'NONE',  ( -5.850000000000018296, 12.50000000000000000, 2.857883832488649301 ) ) ;
#77059=CONICAL_SURFACE ( 'NONE', #5926, 0.09999999999999982514, 0.003490658503988666988 ) ;
#77060=ORIENTED_EDGE ( 'NONE', *, *, #55883, .T. ) ;
#77061=AXIS2_PLACEMENT_3D ( 'NONE', #126447, #36783, #76692 ) ;
#77062=DIRECTION ( 'NONE',  ( 0.000000000000000000, 1.000000000000000000, 0.000000000000000000 ) ) ;
#77063=AXIS2_PLACEMENT_3D ( 'NONE', #9571, #80252, #87466 ) ;
#77064=CIRCLE ( 'NONE', #47832, 0.06509327318403745899 ) ;
#77065=DIRECTION ( 'NONE',  ( 0.000000000000000000, 1.000000000000000000, 0.000000000000000000 ) ) ;
#77066=CARTESIAN_POINT ( 'NONE',  ( 8.349999999999923261, 12.50000000000000000, -7.188010851410854052 ) ) ;
#77067=VERTEX_POINT ( 'NONE', #75774 ) ;
#77068=AXIS2_PLACEMENT_3D ( 'NONE', #108952, #29146, #116848 ) ;
#77069=ORIENTED_EDGE ( 'NONE', *, *, #25911, .T. ) ;
#77070=CONICAL_SURFACE ( 'NONE', #37377, 0.1000000000000002554, 0.003490658503988666988 ) ;
#77071=ORIENTED_EDGE ( 'NONE', *, *, #19772, .F. ) ;
#77072=ORIENTED_EDGE ( 'NONE', *, *, #122180, .T. ) ;
#77075=EDGE_CURVE ( 'NONE', #31468, #53805, #52577, .T. ) ;
#77076=CARTESIAN_POINT ( 'NONE',  ( -1.650000000000035216, 2.500000000000000000, -5.802370205355749988 ) ) ;
#77077=FACE_OUTER_BOUND ( 'NONE', #123066, .T. ) ;
#77078=EDGE_CURVE ( 'NONE', #58403, #38961, #46222, .T. ) ;
#77079=CARTESIAN_POINT ( 'NONE',  ( -13.94999999999998863, 2.500000000000000000, -1.918653347947324006 ) ) ;
#77080=CIRCLE ( 'NONE', #79235, 0.1000000000000002554 ) ;
#77081=ORIENTED_EDGE ( 'NONE', *, *, #120506, .F. ) ;
#77082=ADVANCED_FACE ( 'NONE', ( #24762 ), #69286, .T. ) ;
#77083=FACE_OUTER_BOUND ( 'NONE', #103152, .T. ) ;
#77084=ORIENTED_EDGE ( 'NONE', *, *, #112938, .F. ) ;
#77085=AXIS2_PLACEMENT_3D ( 'NONE', #110688, #91705, #12490 ) ;
#77086=CARTESIAN_POINT ( 'NONE',  ( 76.45351065619851738, -3.568406926262015944, -6.085611129014742993 ) ) ;
#77087=DIRECTION ( 'NONE',  ( 0.000000000000000000, 1.000000000000000000, 0.000000000000000000 ) ) ;
#77088=CARTESIAN_POINT ( 'NONE',  ( 4.999999999999971578, 2.500000000000000000, 0.09999999999999772959 ) ) ;
#77089=CARTESIAN_POINT ( 'NONE',  ( 21.23528140090950700, -2.699413673072311948, 2.293764360948884473 ) ) ;
#77090=ADVANCED_FACE ( 'NONE', ( #77077 ), #10694, .T. ) ;
#77091=EDGE_CURVE ( 'NONE', #72485, #117365, #14886, .T. ) ;
#77092=EDGE_LOOP ( 'NONE', ( #60387, #123249, #46225, #20097 ) ) ;
#77093=EDGE_CURVE ( 'NONE', #25527, #122087, #35856, .T. ) ;
#77094=ADVANCED_FACE ( 'NONE', ( #36527 ), #54221, .T. ) ;
#77095=ORIENTED_EDGE ( 'NONE', *, *, #111776, .F. ) ;
#77096=ORIENTED_EDGE ( 'NONE', *, *, #42936, .T. ) ;
#77097=ORIENTED_EDGE ( 'NONE', *, *, #127317, .T. ) ;
#77098=DIRECTION ( 'NONE',  ( 0.000000000000000000, 1.000000000000000000, 0.000000000000000000 ) ) ;
#77099=CARTESIAN_POINT ( 'NONE',  ( 1.649999999999949729, 2.500000000000000000, 7.288010851410849256 ) ) ;
#77100=FACE_OUTER_BOUND ( 'NONE', #81189, .T. ) ;
#77101=FACE_BOUND ( 'NONE', #64440, .T. ) ;
#77102=LINE ( 'NONE', #35255, #15909 ) ;
#77103=DIRECTION ( 'NONE',  ( 0.000000000000000000, 0.000000000000000000, 1.000000000000000000 ) ) ;
#77104=AXIS2_PLACEMENT_3D ( 'NONE', #128570, #38902, #78812 ) ;
#77105=EDGE_CURVE ( 'NONE', #53767, #76087, #29589, .T. ) ;
#77106=FACE_OUTER_BOUND ( 'NONE', #119344, .T. ) ;
#77107=LINE ( 'NONE', #28003, #70944 ) ;
#77109=DIRECTION ( 'NONE',  ( 0.000000000000000000, 0.000000000000000000, 1.000000000000000000 ) ) ;
#77110=CIRCLE ( 'NONE', #104297, 0.06509327318403745899 ) ;
#77111=CARTESIAN_POINT ( 'NONE',  ( -11.64999999999999680, 12.50000000000000000, 7.188010851410848723 ) ) ;
#77112=DIRECTION ( 'NONE',  ( -0.000000000000000000, 1.000000000000000000, -0.000000000000000000 ) ) ;
#77113=CONICAL_SURFACE ( 'NONE', #52082, 0.1000000000000000472, 0.003490658503988666988 ) ;
#77114=ORIENTED_EDGE ( 'NONE', *, *, #28397, .F. ) ;
#77115=ORIENTED_EDGE ( 'NONE', *, *, #12042, .T. ) ;
#77116=ORIENTED_EDGE ( 'NONE', *, *, #33180, .F. ) ;
#77117=EDGE_LOOP ( 'NONE', ( #61527, #92922, #9084, #14465 ) ) ;
#77118=AXIS2_PLACEMENT_3D ( 'NONE', #95321, #24646, #44936 ) ;
#77119=DIRECTION ( 'NONE',  ( 0.000000000000000000, 1.000000000000000000, 0.000000000000000000 ) ) ;
#77120=ADVANCED_FACE ( 'NONE', ( #84957 ), #124890, .T. ) ;
#77121=FACE_BOUND ( 'NONE', #8820, .T. ) ;
#77122=CARTESIAN_POINT ( 'NONE',  ( -7.500000000000016875, 12.50000000000000000, 0.6928203230275494784 ) ) ;
#77123=DIRECTION ( 'NONE',  ( 0.000000000000000000, 1.000000000000000000, 0.000000000000000000 ) ) ;
#77124=AXIS2_PLACEMENT_3D ( 'NONE', #92825, #73805, #24077 ) ;
#77125=VECTOR ( 'NONE', #3036, 1000.000000000000000 ) ;
#77126=ORIENTED_EDGE ( 'NONE', *, *, #107776, .F. ) ;
#77127=DIRECTION ( 'NONE',  ( -0.000000000000000000, -1.000000000000000000, -0.000000000000000000 ) ) ;
#77128=DIRECTION ( 'NONE',  ( 0.000000000000000000, 1.000000000000000000, 0.000000000000000000 ) ) ;
#77129=ORIENTED_EDGE ( 'NONE', *, *, #76044, .F. ) ;
#77130=CARTESIAN_POINT ( 'NONE',  ( 12.89999999999990266, 2.500000000000000000, -5.122947341949753763 ) ) ;
#77131=DIRECTION ( 'NONE',  ( -0.000000000000000000, -1.000000000000000000, -0.000000000000000000 ) ) ;
#77132=EDGE_CURVE ( 'NONE', #123357, #56703, #75550, .T. ) ;
#77133=ORIENTED_EDGE ( 'NONE', *, *, #53991, .T. ) ;
#77134=AXIS2_PLACEMENT_3D ( 'NONE', #2253, #62500, #98681 ) ;
#77135=CARTESIAN_POINT ( 'NONE',  ( -7.499999999999976907, 12.50000000000000000, 4.330127018922196314 ) ) ;
#77136=CARTESIAN_POINT ( 'NONE',  ( 3.349999999999944578, 2.500000000000000000, -1.372243186433550033 ) ) ;
#77137=EDGE_LOOP ( 'NONE', ( #126305, #4900, #110934, #72087 ) ) ;
#77138=CIRCLE ( 'NONE', #68724, 0.1000000000000000472 ) ;
#77139=CARTESIAN_POINT ( 'NONE',  ( 9.399999999999915090, 2.500000000000000000, -4.676537180435977881 ) ) ;
#77140=VECTOR ( 'NONE', #50322, 1000.000000000000000 ) ;
#77141=DIRECTION ( 'NONE',  ( 0.000000000000000000, 0.000000000000000000, 1.000000000000000000 ) ) ;
#77142=ORIENTED_EDGE ( 'NONE', *, *, #114763, .F. ) ;
#77143=PLANE ( 'NONE',  #93273 ) ;
#77144=ORIENTED_EDGE ( 'NONE', *, *, #81081, .T. ) ;
#77145=ORIENTED_EDGE ( 'NONE', *, *, #71021, .T. ) ;
#77147=CARTESIAN_POINT ( 'NONE',  ( 7.899999999999924860, 2.500000000000000000, 3.637306695894644726 ) ) ;
#77148=EDGE_LOOP ( 'NONE', ( #115038, #111109 ) ) ;
#77149=DIRECTION ( 'NONE',  ( 0.000000000000000000, 1.000000000000000000, 0.000000000000000000 ) ) ;
#77150=FACE_BOUND ( 'NONE', #61922, .T. ) ;
#77151=CONICAL_SURFACE ( 'NONE', #54176, 0.09999999999999982514, 0.003490658503988666988 ) ;
#77153=VERTEX_POINT ( 'NONE', #46985 ) ;
#77155=VERTEX_POINT ( 'NONE', #65961 ) ;
#77156=CARTESIAN_POINT ( 'NONE',  ( -4.150000000000025224, 2.500000000000000000, 2.957883832488649389 ) ) ;
#77157=DIRECTION ( 'NONE',  ( 0.000000000000000000, 1.000000000000000000, 0.000000000000000000 ) ) ;
#77158=DIRECTION ( 'NONE',  ( 0.000000000000000000, 0.000000000000000000, 1.000000000000000000 ) ) ;
#77159=DIRECTION ( 'NONE',  ( 0.000000000000000000, -0.9999939076577903929, 0.003490651415223739937 ) ) ;
#77160=CARTESIAN_POINT ( 'NONE',  ( 7.099999999999926814, 2.500000000000000000, -0.1000000000000022815 ) ) ;
#77161=CIRCLE ( 'NONE', #75109, 0.06509327318403745899 ) ;
#77162=ORIENTED_EDGE ( 'NONE', *, *, #20632, .F. ) ;
#77163=AXIS2_PLACEMENT_3D ( 'NONE', #112481, #30714, #110534 ) ;
#77164=VERTEX_POINT ( 'NONE', #86886 ) ;
#77165=DIRECTION ( 'NONE',  ( -0.000000000000000000, 1.000000000000000000, -0.000000000000000000 ) ) ;
#77166=DIRECTION ( 'NONE',  ( 0.000000000000000000, 1.000000000000000000, 0.000000000000000000 ) ) ;
#77167=FACE_OUTER_BOUND ( 'NONE', #117568, .T. ) ;
#77168=ORIENTED_EDGE ( 'NONE', *, *, #4218, .T. ) ;
#77169=ORIENTED_EDGE ( 'NONE', *, *, #31744, .T. ) ;
#77170=ORIENTED_EDGE ( 'NONE', *, *, #40470, .T. ) ;
#77171=CARTESIAN_POINT ( 'NONE',  ( -5.450000000000019718, 2.500000000000000000, 6.395190528383296602 ) ) ;
#77172=DIRECTION ( 'NONE',  ( -4.274815082592931898E-19, -0.9999939076577903929, -0.003490651415223739937 ) ) ;
#77173=LINE ( 'NONE', #112284, #5976 ) ;
#77174=EDGE_CURVE ( 'NONE', #28403, #31157, #54841, .T. ) ;
#77176=DIRECTION ( 'NONE',  ( 0.000000000000000000, 0.000000000000000000, 1.000000000000000000 ) ) ;
#77177=CARTESIAN_POINT ( 'NONE',  ( -12.69999999999999396, 2.500000000000000000, 0.4464101615137776591 ) ) ;
#77178=DIRECTION ( 'NONE',  ( -0.000000000000000000, 1.000000000000000000, -0.000000000000000000 ) ) ;
#77179=DIRECTION ( 'NONE',  ( -0.000000000000000000, 1.000000000000000000, -0.000000000000000000 ) ) ;
#77180=CIRCLE ( 'NONE', #127361, 0.06509327318403745899 ) ;
#77181=DIRECTION ( 'NONE',  ( -0.000000000000000000, 1.000000000000000000, -0.000000000000000000 ) ) ;
#77182=DIRECTION ( 'NONE',  ( 0.000000000000000000, 1.000000000000000000, 0.000000000000000000 ) ) ;
#77183=ADVANCED_FACE ( 'NONE', ( #94782 ), #75146, .T. ) ;
#77184=VERTEX_POINT ( 'NONE', #55508 ) ;
#77185=VERTEX_POINT ( 'NONE', #67214 ) ;
#77186=PLANE ( 'NONE',  #65363 ) ;
#77187=EDGE_CURVE ( 'NONE', #83854, #6221, #97356, .T. ) ;
#77188=ORIENTED_EDGE ( 'NONE', *, *, #95663, .T. ) ;
#77189=ADVANCED_FACE ( 'NONE', ( #109764 ), #39114, .T. ) ;
#77190=ORIENTED_EDGE ( 'NONE', *, *, #65340, .T. ) ;
#77191=EDGE_CURVE ( 'NONE', #67175, #63506, #8322, .T. ) ;
#77192=DIRECTION ( 'NONE',  ( 0.000000000000000000, 0.000000000000000000, 1.000000000000000000 ) ) ;
#77193=CARTESIAN_POINT ( 'NONE',  ( 97.50000000000000000, 0.000000000000000000, 0.000000000000000000 ) ) ;
#77194=ADVANCED_FACE ( 'NONE', ( #29276 ), #17491, .T. ) ;
#77195=AXIS2_PLACEMENT_3D ( 'NONE', #37439, #77349, #117239 ) ;
#77196=LINE ( 'NONE', #117094, #67542 ) ;
#77198=LINE ( 'NONE', #115824, #2607 ) ;
#77199=CARTESIAN_POINT ( 'NONE',  ( 10.79999999999991012, 2.500000000000000000, -4.330127018922201643 ) ) ;
#77200=DIRECTION ( 'NONE',  ( 0.000000000000000000, 0.000000000000000000, -1.000000000000000000 ) ) ;
#77201=ORIENTED_EDGE ( 'NONE', *, *, #21058, .T. ) ;
#77202=DIRECTION ( 'NONE',  ( -4.274815082592931898E-19, -0.9999939076577903929, -0.003490651415223739937 ) ) ;
#77203=ADVANCED_FACE ( 'NONE', ( #57441 ), #8963, .T. ) ;
#77204=DIRECTION ( 'NONE',  ( -0.000000000000000000, -1.000000000000000000, -0.000000000000000000 ) ) ;
#77205=EDGE_CURVE ( 'NONE', #58364, #88434, #12840, .T. ) ;
#77206=EDGE_CURVE ( 'NONE', #112593, #10182, #33705, .T. ) ;
#77207=ORIENTED_EDGE ( 'NONE', *, *, #69047, .T. ) ;
#77208=CIRCLE ( 'NONE', #14480, 0.1000000000000000472 ) ;
#77209=CIRCLE ( 'NONE', #93934, 0.1000000000000002554 ) ;
#77210=ORIENTED_EDGE ( 'NONE', *, *, #34808, .F. ) ;
#77211=AXIS2_PLACEMENT_3D ( 'NONE', #14008, #53955, #122059 ) ;
#77212=ORIENTED_EDGE ( 'NONE', *, *, #116223, .T. ) ;
#77213=EDGE_LOOP ( 'NONE', ( #116592, #84251 ) ) ;
#77214=DIRECTION ( 'NONE',  ( -0.000000000000000000, 1.000000000000000000, -0.000000000000000000 ) ) ;
#77215=CARTESIAN_POINT ( 'NONE',  ( 5.649999999999934630, 2.500000000000000000, 6.841600689897072485 ) ) ;
#77216=VECTOR ( 'NONE', #97324, 1000.000000000000000 ) ;
#77217=AXIS2_PLACEMENT_3D ( 'NONE', #62606, #54676, #81581 ) ;
#77218=VERTEX_POINT ( 'NONE', #47621 ) ;
#77219=DIRECTION ( 'NONE',  ( 0.000000000000000000, 0.000000000000000000, -1.000000000000000000 ) ) ;
#77220=CARTESIAN_POINT ( 'NONE',  ( 17.50000000000000000, 2.749999999999999556, -9.999999999999998224 ) ) ;
#77221=CARTESIAN_POINT ( 'NONE',  ( -9.150000000000005684, 12.50000000000000000, 7.253104124594885960 ) ) ;
#77222=ORIENTED_EDGE ( 'NONE', *, *, #106424, .F. ) ;
#77223=DIRECTION ( 'NONE',  ( 0.000000000000000000, 0.000000000000000000, 1.000000000000000000 ) ) ;
#77224=DIRECTION ( 'NONE',  ( -0.000000000000000000, -1.000000000000000000, -0.000000000000000000 ) ) ;
#77225=VERTEX_POINT ( 'NONE', #28630 ) ;
#77226=EDGE_LOOP ( 'NONE', ( #119622, #41907, #107734, #64328 ) ) ;
#77227=ORIENTED_EDGE ( 'NONE', *, *, #21441, .T. ) ;
#77228=CARTESIAN_POINT ( 'NONE',  ( 12.93920187831545299, -1.499999999999998446, 10.00000000000000178 ) ) ;
#77229=CARTESIAN_POINT ( 'NONE',  ( 1.649999999999951505, 2.500000000000000000, -1.572243186433550211 ) ) ;
#77230=CONICAL_SURFACE ( 'NONE', #66847, 0.1000000000000002554, 0.003490658503988666988 ) ;
#77231=VECTOR ( 'NONE', #46286, 1000.000000000000000 ) ;
#77232=ORIENTED_EDGE ( 'NONE', *, *, #15703, .F. ) ;
#77233=PLANE ( 'NONE',  #11942 ) ;
#77234=CARTESIAN_POINT ( 'NONE',  ( -6.250000000000017764, 12.50000000000000000, 2.857883832488649301 ) ) ;
#77235=DIRECTION ( 'NONE',  ( 0.000000000000000000, 0.000000000000000000, -1.000000000000000000 ) ) ;
#77236=CARTESIAN_POINT ( 'NONE',  ( -5.000000000000026645, 2.500000000000000000, -3.637306695894650055 ) ) ;
#77237=EDGE_CURVE ( 'NONE', #104608, #75247, #29508, .T. ) ;
#77238=AXIS2_PLACEMENT_3D ( 'NONE', #127138, #126485, #86548 ) ;
#77239=CONICAL_SURFACE ( 'NONE', #62587, 0.1000000000000002554, 0.003490658503988666988 ) ;
#77240=EDGE_CURVE ( 'NONE', #13780, #100057, #99302, .T. ) ;
#77242=AXIS2_PLACEMENT_3D ( 'NONE', #102749, #43863, #81199 ) ;
#77243=CARTESIAN_POINT ( 'NONE',  ( 12.09999999999990550, 2.500000000000000000, -4.430127018922202176 ) ) ;
#77244=ADVANCED_FACE ( 'NONE', ( #118932 ), #6475, .T. ) ;
#77245=ORIENTED_EDGE ( 'NONE', *, *, #101497, .F. ) ;
#77246=EDGE_LOOP ( 'NONE', ( #120721, #29660 ) ) ;
#77247=CARTESIAN_POINT ( 'NONE',  ( 3.149999999999946176, 12.50000000000000000, -6.841600689897077814 ) ) ;
#77249=CARTESIAN_POINT ( 'NONE',  ( 4.999999999999935163, 2.500000000000000000, 0.5928203230275495006 ) ) ;
#77250=FACE_BOUND ( 'NONE', #70593, .T. ) ;
#77251=VECTOR ( 'NONE', #104777, 1000.000000000000000 ) ;
#77252=DIRECTION ( 'NONE',  ( 0.000000000000000000, 0.000000000000000000, 1.000000000000000000 ) ) ;
#77253=CARTESIAN_POINT ( 'NONE',  ( -3.150000000000032330, 12.50000000000000000, -6.148780366869526226 ) ) ;
#77254=EDGE_CURVE ( 'NONE', #28344, #102426, #106846, .T. ) ;
#77255=DIRECTION ( 'NONE',  ( 0.000000000000000000, 0.000000000000000000, -1.000000000000000000 ) ) ;
#77256=CIRCLE ( 'NONE', #79332, 0.06509327318403745899 ) ;
#77257=AXIS2_PLACEMENT_3D ( 'NONE', #78718, #78052, #49258 ) ;
#77258=ORIENTED_EDGE ( 'NONE', *, *, #38222, .F. ) ;
#77259=DIRECTION ( 'NONE',  ( 0.000000000000000000, -0.9999939076577903929, 0.003490651415223739937 ) ) ;
#77260=FACE_OUTER_BOUND ( 'NONE', #41036, .T. ) ;
#77261=CARTESIAN_POINT ( 'NONE',  ( 6.849999999999929479, 2.500000000000000000, -2.611473670974877592 ) ) ;
#77262=CARTESIAN_POINT ( 'NONE',  ( 12.94999999999990337, 2.500000000000000000, 2.265063509461097357 ) ) ;
#77263=ORIENTED_EDGE ( 'NONE', *, *, #112585, .T. ) ;
#77264=DIRECTION ( 'NONE',  ( 0.000000000000000000, 1.000000000000000000, 0.000000000000000000 ) ) ;
#77265=DIRECTION ( 'NONE',  ( -4.274815082592931898E-19, -0.9999939076577903929, -0.003490651415223739937 ) ) ;
#77266=AXIS2_PLACEMENT_3D ( 'NONE', #53815, #21799, #93749 ) ;
#77267=ORIENTED_EDGE ( 'NONE', *, *, #6202, .F. ) ;
#77268=DIRECTION ( 'NONE',  ( 0.000000000000000000, 0.000000000000000000, -1.000000000000000000 ) ) ;
#77269=DIRECTION ( 'NONE',  ( 0.000000000000000000, 1.000000000000000000, 0.000000000000000000 ) ) ;
#77270=EDGE_CURVE ( 'NONE', #42494, #43342, #44166, .T. ) ;
#77271=FACE_BOUND ( 'NONE', #107243, .T. ) ;
#77272=CARTESIAN_POINT ( 'NONE',  ( -15.59999999999998010, 2.500000000000000000, 0.2464101615137759549 ) ) ;
#77273=ORIENTED_EDGE ( 'NONE', *, *, #74083, .F. ) ;
#77274=DIRECTION ( 'NONE',  ( 0.000000000000000000, 0.000000000000000000, 1.000000000000000000 ) ) ;
#77275=ORIENTED_EDGE ( 'NONE', *, *, #47964, .F. ) ;
#77276=ORIENTED_EDGE ( 'NONE', *, *, #29246, .F. ) ;
#77277=CARTESIAN_POINT ( 'NONE',  ( 11.64999999999990443, 2.500000000000000000, -5.802370205355749988 ) ) ;
#77279=ORIENTED_EDGE ( 'NONE', *, *, #118124, .F. ) ;
#77280=CARTESIAN_POINT ( 'NONE',  ( 11.84999999999990727, 2.500000000000000000, -1.718653347947326049 ) ) ;
#77281=CARTESIAN_POINT ( 'NONE',  ( 11.84999999999990372, 12.50000000000000000, 1.753560074763284016 ) ) ;
#77282=EDGE_CURVE ( 'NONE', #98143, #63986, #119376, .T. ) ;
#77283=PLANE ( 'NONE',  #119668 ) ;
#77285=ORIENTED_EDGE ( 'NONE', *, *, #86837, .T. ) ;
#77286=CARTESIAN_POINT ( 'NONE',  ( -7.900000000000014566, 12.50000000000000000, 0.6928203230275494784 ) ) ;
#77287=VECTOR ( 'NONE', #93967, 1000.000000000000000 ) ;
#77289=CARTESIAN_POINT ( 'NONE',  ( -5.650000000000023448, 2.500000000000000000, -6.048780366869526581 ) ) ;
#77290=DIRECTION ( 'NONE',  ( -0.000000000000000000, -1.000000000000000000, -0.000000000000000000 ) ) ;
#77291=CARTESIAN_POINT ( 'NONE',  ( 16.55712575656180618, -0.2764121571830139845, -6.093697237267636346 ) ) ;
#77292=AXIS2_PLACEMENT_3D ( 'NONE', #88557, #99034, #99688 ) ;
#77293=EDGE_LOOP ( 'NONE', ( #91783, #98055 ) ) ;
#77294=FACE_OUTER_BOUND ( 'NONE', #115526, .T. ) ;
#77295=ORIENTED_EDGE ( 'NONE', *, *, #95769, .F. ) ;
#77296=EDGE_CURVE ( 'NONE', #91497, #50580, #116978, .T. ) ;
#77297=CARTESIAN_POINT ( 'NONE',  ( 3.549999999999944755, 2.500000000000000000, -2.511473670974877948 ) ) ;
#77298=CARTESIAN_POINT ( 'NONE',  ( 10.84999999999991260, 2.500000000000000000, 7.188010851410848723 ) ) ;
#77299=ORIENTED_EDGE ( 'NONE', *, *, #43622, .F. ) ;
#77300=CARTESIAN_POINT ( 'NONE',  ( -3.150000000000030109, 2.500000000000000000, -2.611473670974877592 ) ) ;
#77301=VECTOR ( 'NONE', #100397, 1000.000000000000000 ) ;
#77302=VECTOR ( 'NONE', #52446, 1000.000000000000000 ) ;
#77303=DIRECTION ( 'NONE',  ( 0.000000000000000000, -0.000000000000000000, 1.000000000000000000 ) ) ;
#77304=LINE ( 'NONE', #97583, #66343 ) ;
#77305=DIRECTION ( 'NONE',  ( 0.000000000000000000, 1.000000000000000000, 0.000000000000000000 ) ) ;
#77306=ORIENTED_EDGE ( 'NONE', *, *, #37633, .T. ) ;
#77307=CARTESIAN_POINT ( 'NONE',  ( 5.649999999999934630, 2.500000000000000000, 6.841600689897072485 ) ) ;
#77308=CARTESIAN_POINT ( 'NONE',  ( -4.600000000000028066, 2.500000000000000000, -4.922947341949753586 ) ) ;
#77309=ADVANCED_FACE ( 'NONE', ( #49564 ), #79675, .T. ) ;
#77310=DIRECTION ( 'NONE',  ( -0.000000000000000000, 1.000000000000000000, -0.000000000000000000 ) ) ;
#77311=CARTESIAN_POINT ( 'NONE',  ( 1.649999999999949729, 2.500000000000000000, 7.188010851410848723 ) ) ;
#77312=CARTESIAN_POINT ( 'NONE',  ( -11.64999999999999680, 2.500000000000000000, 6.495190528383297135 ) ) ;
#77313=VERTEX_POINT ( 'NONE', #18145 ) ;
#77314=ORIENTED_EDGE ( 'NONE', *, *, #54206, .F. ) ;
#77315=DIRECTION ( 'NONE',  ( -0.000000000000000000, 1.000000000000000000, -0.000000000000000000 ) ) ;
#77316=ORIENTED_EDGE ( 'NONE', *, *, #16994, .T. ) ;
#77317=PLANE ( 'NONE',  #97979 ) ;
#77318=ORIENTED_EDGE ( 'NONE', *, *, #2770, .F. ) ;
#77319=EDGE_LOOP ( 'NONE', ( #75200, #123005, #71835, #43835 ) ) ;
#77320=ORIENTED_EDGE ( 'NONE', *, *, #80922, .T. ) ;
#77321=CARTESIAN_POINT ( 'NONE',  ( -10.65000000000000391, 12.50000000000000000, -2.511473670974873951 ) ) ;
#77322=CONICAL_SURFACE ( 'NONE', #98148, 0.1000000000000002554, 0.003490658503988666988 ) ;
#77323=CARTESIAN_POINT ( 'NONE',  ( 1.649999999999951505, 2.500000000000000000, -2.757883832488654097 ) ) ;
#77324=AXIS2_PLACEMENT_3D ( 'NONE', #24504, #95177, #53965 ) ;
#77325=CARTESIAN_POINT ( 'NONE',  ( -4.400000000000025224, 2.500000000000000000, 4.576537180435972019 ) ) ;
#77326=EDGE_CURVE ( 'NONE', #33696, #116195, #58091, .T. ) ;
#77328=DIRECTION ( 'NONE',  ( 0.000000000000000000, 0.000000000000000000, 1.000000000000000000 ) ) ;
#77329=CARTESIAN_POINT ( 'NONE',  ( 1.449999999999952216, 12.50000000000000000, -2.511473670974877948 ) ) ;
#77330=DIRECTION ( 'NONE',  ( 0.000000000000000000, 1.000000000000000000, 0.000000000000000000 ) ) ;
#77331=DIRECTION ( 'NONE',  ( 0.000000000000000000, 0.000000000000000000, -1.000000000000000000 ) ) ;
#77332=ORIENTED_EDGE ( 'NONE', *, *, #72486, .F. ) ;
#77333=DIRECTION ( 'NONE',  ( 0.000000000000000000, 0.000000000000000000, -1.000000000000000000 ) ) ;
#77335=ORIENTED_EDGE ( 'NONE', *, *, #48388, .T. ) ;
#77336=EDGE_CURVE ( 'NONE', #116085, #31429, #19099, .T. ) ;
#77337=ORIENTED_EDGE ( 'NONE', *, *, #68048, .T. ) ;
#77338=EDGE_LOOP ( 'NONE', ( #59322, #127813 ) ) ;
#77339=ORIENTED_EDGE ( 'NONE', *, *, #60532, .F. ) ;
#77340=CARTESIAN_POINT ( 'NONE',  ( -4.200000000000025935, 12.50000000000000000, 4.330127018922196314 ) ) ;
#77341=ADVANCED_FACE ( 'NONE', ( #30575 ), #37908, .T. ) ;
#77342=ORIENTED_EDGE ( 'NONE', *, *, #75812, .F. ) ;
#77343=ADVANCED_FACE ( 'NONE', ( #61954 ), #96383, .T. ) ;
#77344=VERTEX_POINT ( 'NONE', #82888 ) ;
#77345=EDGE_CURVE ( 'NONE', #47774, #110068, #127790, .T. ) ;
#77346=CIRCLE ( 'NONE', #127520, 0.1000000000000000472 ) ;
#77347=EDGE_CURVE ( 'NONE', #42074, #55928, #52764, .T. ) ;
#77348=DIRECTION ( 'NONE',  ( -0.000000000000000000, 1.000000000000000000, -0.000000000000000000 ) ) ;
#77349=DIRECTION ( 'NONE',  ( -0.000000000000000000, 1.000000000000000000, -0.000000000000000000 ) ) ;
#77350=CIRCLE ( 'NONE', #18846, 0.06509327318403745899 ) ;
#77352=DIRECTION ( 'NONE',  ( 0.000000000000000000, 0.000000000000000000, 1.000000000000000000 ) ) ;
#77353=CARTESIAN_POINT ( 'NONE',  ( 4.999999999999938716, 2.500000000000000000, -5.122947341949753763 ) ) ;
#77355=DIRECTION ( 'NONE',  ( 0.000000000000000000, 0.000000000000000000, 1.000000000000000000 ) ) ;
#77356=VERTEX_POINT ( 'NONE', #20736 ) ;
#77357=EDGE_CURVE ( 'NONE', #53692, #12100, #2478, .T. ) ;
#77358=AXIS2_PLACEMENT_3D ( 'NONE', #27542, #98230, #107412 ) ;
#77359=CARTESIAN_POINT ( 'NONE',  ( 6.649999999999931077, 12.50000000000000000, -6.495190528383302464 ) ) ;
#77360=AXIS2_PLACEMENT_3D ( 'NONE', #54375, #56305, #104747 ) ;
#77361=EDGE_CURVE ( 'NONE', #74772, #113119, #81580, .T. ) ;
#77362=ORIENTED_EDGE ( 'NONE', *, *, #77036, .F. ) ;
#77363=CARTESIAN_POINT ( 'NONE',  ( 8.749999999999921840, 12.50000000000000000, -5.802370205355749988 ) ) ;
#77364=EDGE_CURVE ( 'NONE', #4623, #125419, #121489, .T. ) ;
#77365=EDGE_LOOP ( 'NONE', ( #59052, #21160 ) ) ;
#77366=CARTESIAN_POINT ( 'NONE',  ( 2.699999999999946443, 2.500000000000000000, 0.2464101615137735679 ) ) ;
#77367=CIRCLE ( 'NONE', #98277, 0.06509327318403745899 ) ;
#77368=VERTEX_POINT ( 'NONE', #111019 ) ;
#77369=ORIENTED_EDGE ( 'NONE', *, *, #16609, .T. ) ;
#77370=EDGE_CURVE ( 'NONE', #33550, #100266, #50842, .T. ) ;
#77371=DIRECTION ( 'NONE',  ( 0.000000000000000000, 0.000000000000000000, -1.000000000000000000 ) ) ;
#77372=CARTESIAN_POINT ( 'NONE',  ( 6.699999999999930012, 12.50000000000000000, -4.330127018922201643 ) ) ;
#77374=CARTESIAN_POINT ( 'NONE',  ( 13.54999999999989591, 12.50000000000000000, -1.818653347947326138 ) ) ;
#77375=DIRECTION ( 'NONE',  ( -0.000000000000000000, -1.000000000000000000, -0.000000000000000000 ) ) ;
#77376=VERTEX_POINT ( 'NONE', #72420 ) ;
#77377=DIRECTION ( 'NONE',  ( 0.000000000000000000, -0.9999939076577903929, 0.003490651415223739937 ) ) ;
#77378=DIRECTION ( 'NONE',  ( 0.000000000000000000, 0.000000000000000000, -1.000000000000000000 ) ) ;
#77380=DIRECTION ( 'NONE',  ( 0.000000000000000000, 1.000000000000000000, 0.000000000000000000 ) ) ;
#77381=LINE ( 'NONE', #15205, #70977 ) ;
#77382=EDGE_LOOP ( 'NONE', ( #96348, #61239, #5035, #57690 ) ) ;
#77383=ORIENTED_EDGE ( 'NONE', *, *, #42840, .F. ) ;
#77384=VECTOR ( 'NONE', #40981, 1000.000000000000000 ) ;
#77385=DIRECTION ( 'NONE',  ( 0.000000000000000000, 1.000000000000000000, 0.000000000000000000 ) ) ;
#77386=CIRCLE ( 'NONE', #92042, 0.1000000000000000472 ) ;
#77387=ORIENTED_EDGE ( 'NONE', *, *, #117414, .F. ) ;
#77388=DIRECTION ( 'NONE',  ( 0.000000000000000000, 0.000000000000000000, 1.000000000000000000 ) ) ;
#77389=CARTESIAN_POINT ( 'NONE',  ( -11.25000000000000000, 2.500000000000000000, 2.857883832488649301 ) ) ;
#77390=CONICAL_SURFACE ( 'NONE', #16807, 0.1000000000000000472, 0.003490658503988666988 ) ;
#77391=CIRCLE ( 'NONE', #20951, 0.06509327318403745899 ) ;
#77392=ORIENTED_EDGE ( 'NONE', *, *, #26473, .T. ) ;
#77394=DIRECTION ( 'NONE',  ( 0.000000000000000000, 0.000000000000000000, 1.000000000000000000 ) ) ;
#77395=FACE_OUTER_BOUND ( 'NONE', #105733, .T. ) ;
#77396=DIRECTION ( 'NONE',  ( 0.000000000000000000, 1.000000000000000000, 0.000000000000000000 ) ) ;
#77397=ORIENTED_EDGE ( 'NONE', *, *, #50922, .F. ) ;
#77398=AXIS2_PLACEMENT_3D ( 'NONE', #6661, #67529, #126483 ) ;
#77399=EDGE_CURVE ( 'NONE', #61052, #29513, #52135, .T. ) ;
#77400=DIRECTION ( 'NONE',  ( 0.000000000000000000, 0.000000000000000000, 1.000000000000000000 ) ) ;
#77402=ADVANCED_FACE ( 'NONE', ( #1723 ), #82239, .T. ) ;
#77403=ORIENTED_EDGE ( 'NONE', *, *, #76206, .T. ) ;
#77404=DIRECTION ( 'NONE',  ( 0.000000000000000000, -0.000000000000000000, 1.000000000000000000 ) ) ;
#77405=DIRECTION ( 'NONE',  ( 0.000000000000000000, 0.000000000000000000, -1.000000000000000000 ) ) ;
#77406=CARTESIAN_POINT ( 'NONE',  ( -1.850000000000033840, 2.500000000000000000, 1.718653347947321386 ) ) ;
#77407=EDGE_CURVE ( 'NONE', #96594, #60331, #81900, .T. ) ;
#77408=VERTEX_POINT ( 'NONE', #60673 ) ;
#77409=CARTESIAN_POINT ( 'NONE',  ( -7.100000000000013856, 12.50000000000000000, 5.022947341949748790 ) ) ;
#77410=ORIENTED_EDGE ( 'NONE', *, *, #81342, .T. ) ;
#77411=DIRECTION ( 'NONE',  ( 0.000000000000000000, -0.9999939076577903929, 0.003490651415223739937 ) ) ;
#77412=DIRECTION ( 'NONE',  ( 0.000000000000000000, 1.000000000000000000, 0.000000000000000000 ) ) ;
#77413=PLANE ( 'NONE',  #24539 ) ;
#77415=CIRCLE ( 'NONE', #52289, 0.1000000000000000472 ) ;
#77416=DIRECTION ( 'NONE',  ( -0.000000000000000000, -1.000000000000000000, -0.000000000000000000 ) ) ;
#77417=AXIS2_PLACEMENT_3D ( 'NONE', #14217, #113736, #3772 ) ;
#77418=DIRECTION ( 'NONE',  ( 0.000000000000000000, 0.000000000000000000, -1.000000000000000000 ) ) ;
#77419=ORIENTED_EDGE ( 'NONE', *, *, #9592, .T. ) ;
#77420=LINE ( 'NONE', #27654, #21748 ) ;
#77421=ORIENTED_EDGE ( 'NONE', *, *, #122553, .F. ) ;
#77422=CONICAL_SURFACE ( 'NONE', #12569, 0.1000000000000000472, 0.003490658503988666988 ) ;
#77423=DIRECTION ( 'NONE',  ( 0.000000000000000000, -0.9999939076577903929, 0.003490651415223739937 ) ) ;
#77424=VERTEX_POINT ( 'NONE', #122169 ) ;
#77425=DIRECTION ( 'NONE',  ( 0.000000000000000000, 0.000000000000000000, -1.000000000000000000 ) ) ;
#77426=DIRECTION ( 'NONE',  ( 0.000000000000000000, 0.000000000000000000, -1.000000000000000000 ) ) ;
#77427=ORIENTED_EDGE ( 'NONE', *, *, #106971, .F. ) ;
#77428=EDGE_LOOP ( 'NONE', ( #107988, #60282 ) ) ;
#77429=DIRECTION ( 'NONE',  ( 0.000000000000000000, 1.000000000000000000, 0.000000000000000000 ) ) ;
#77430=DIRECTION ( 'NONE',  ( -0.000000000000000000, 1.000000000000000000, -0.000000000000000000 ) ) ;
#77431=VERTEX_POINT ( 'NONE', #71772 ) ;
#77432=CIRCLE ( 'NONE', #104617, 0.06509327318403745899 ) ;
#77433=CARTESIAN_POINT ( 'NONE',  ( 4.149999999999939959, 12.50000000000000000, 1.472243186433545459 ) ) ;
#77435=CARTESIAN_POINT ( 'NONE',  ( 5.799999999999931433, 2.500000000000000000, 4.330127018922196314 ) ) ;
#77436=VECTOR ( 'NONE', #95450, 1000.000000000000000 ) ;
#77437=DIRECTION ( 'NONE',  ( 0.000000000000000000, -0.9999939076577903929, 0.003490651415223739937 ) ) ;
#77439=CARTESIAN_POINT ( 'NONE',  ( -4.400000000000028777, 2.500000000000000000, -4.676537180435978769 ) ) ;
#77440=DIRECTION ( 'NONE',  ( -4.274815082592931898E-19, -0.9999939076577903929, -0.003490651415223739937 ) ) ;
#77441=AXIS2_PLACEMENT_3D ( 'NONE', #93517, #41216, #102051 ) ;
#77442=ORIENTED_EDGE ( 'NONE', *, *, #65948, .F. ) ;
#77443=EDGE_LOOP ( 'NONE', ( #31440, #21695 ) ) ;
#77444=EDGE_LOOP ( 'NONE', ( #107313, #18190 ) ) ;
#77445=ORIENTED_EDGE ( 'NONE', *, *, #43491, .F. ) ;
#77446=CONICAL_SURFACE ( 'NONE', #27269, 0.1000000000000002554, 0.003490658503988666988 ) ;
#77447=DIRECTION ( 'NONE',  ( 0.000000000000000000, 0.000000000000000000, -1.000000000000000000 ) ) ;
#77448=DIRECTION ( 'NONE',  ( 0.000000000000000000, 0.000000000000000000, -1.000000000000000000 ) ) ;
#77449=ADVANCED_FACE ( 'NONE', ( #112339 ), #62604, .T. ) ;
#77450=DIRECTION ( 'NONE',  ( 0.000000000000000000, 1.000000000000000000, 0.000000000000000000 ) ) ;
#77451=VERTEX_POINT ( 'NONE', #102513 ) ;
#77452=FACE_BOUND ( 'NONE', #57335, .T. ) ;
#77453=ORIENTED_EDGE ( 'NONE', *, *, #5057, .T. ) ;
#77454=DIRECTION ( 'NONE',  ( -0.000000000000000000, -1.000000000000000000, -0.000000000000000000 ) ) ;
#77455=LINE ( 'NONE', #117342, #96075 ) ;
#77456=CARTESIAN_POINT ( 'NONE',  ( -4.400000000000025224, 2.500000000000000000, 3.983716857408420076 ) ) ;
#77457=CARTESIAN_POINT ( 'NONE',  ( 12.69999999999989804, 2.500000000000000000, 0.4464101615137735513 ) ) ;
#77458=CARTESIAN_POINT ( 'NONE',  ( -13.54999999999998828, 2.500000000000000000, -2.611473670974875372 ) ) ;
#77459=LINE ( 'NONE', #127848, #97759 ) ;
#77460=CARTESIAN_POINT ( 'NONE',  ( -5.400000000000020783, 12.50000000000000000, 0.6928203230275494784 ) ) ;
#77461=CARTESIAN_POINT ( 'NONE',  ( 4.149999999999941735, 2.500000000000000000, -7.188010851410854052 ) ) ;
#77462=ADVANCED_FACE ( 'NONE', ( #12816 ), #35946, .T. ) ;
#77463=CARTESIAN_POINT ( 'NONE',  ( 11.44999999999991047, 12.50000000000000000, 6.148780366869520009 ) ) ;
#77464=FACE_OUTER_BOUND ( 'NONE', #70721, .T. ) ;
#77465=ORIENTED_EDGE ( 'NONE', *, *, #23607, .F. ) ;
#77466=VERTEX_POINT ( 'NONE', #112976 ) ;
#77467=ORIENTED_EDGE ( 'NONE', *, *, #807, .T. ) ;
#77468=ORIENTED_EDGE ( 'NONE', *, *, #117163, .F. ) ;
#77469=CARTESIAN_POINT ( 'NONE',  ( 0.4499999999999569344, 12.50000000000000000, -2.230156782645139391 ) ) ;
#77470=CIRCLE ( 'NONE', #98385, 0.1000000000000000472 ) ;
#77471=CARTESIAN_POINT ( 'NONE',  ( -2.100000000000033396, 12.50000000000000000, -3.572213422710612374 ) ) ;
#77472=CIRCLE ( 'NONE', #6421, 0.1000000000000002554 ) ;
#77473=EDGE_LOOP ( 'NONE', ( #19002, #109536 ) ) ;
#77474=ORIENTED_EDGE ( 'NONE', *, *, #15834, .T. ) ;
#77475=VERTEX_POINT ( 'NONE', #13474 ) ;
#77476=CARTESIAN_POINT ( 'NONE',  ( 2.099999999999950351, 2.500000000000000000, -0.1000000000000022815 ) ) ;
#77477=VECTOR ( 'NONE', #47298, 1000.000000000000000 ) ;
#77478=CARTESIAN_POINT ( 'NONE',  ( -10.60000000000000142, 2.500000000000000000, 0.2464101615137736789 ) ) ;
#77479=DIRECTION ( 'NONE',  ( 0.000000000000000000, 0.000000000000000000, 1.000000000000000000 ) ) ;
#77480=FACE_OUTER_BOUND ( 'NONE', #98787, .T. ) ;
#77481=DIRECTION ( 'NONE',  ( 0.000000000000000000, 1.000000000000000000, 0.000000000000000000 ) ) ;
#77483=ORIENTED_EDGE ( 'NONE', *, *, #121679, .T. ) ;
#77484=CARTESIAN_POINT ( 'NONE',  ( 2.949999999999943334, 2.500000000000000000, 6.595190528383296780 ) ) ;
#77485=VERTEX_POINT ( 'NONE', #53427 ) ;
#77486=ADVANCED_FACE ( 'NONE', ( #90756 ), #6223, .T. ) ;
#77487=ORIENTED_EDGE ( 'NONE', *, *, #93046, .F. ) ;
#77488=VERTEX_POINT ( 'NONE', #66448 ) ;
#77489=DIRECTION ( 'NONE',  ( 0.000000000000000000, 0.000000000000000000, 1.000000000000000000 ) ) ;
#77490=VERTEX_POINT ( 'NONE', #65800 ) ;
#77491=EDGE_CURVE ( 'NONE', #67278, #17990, #103808, .T. ) ;
#77492=VERTEX_POINT ( 'NONE', #5579 ) ;
#77493=ADVANCED_FACE ( 'NONE', ( #96536 ), #44227, .T. ) ;
#77494=CARTESIAN_POINT ( 'NONE',  ( -6.850000000000017408, 2.500000000000000000, -1.818653347947325916 ) ) ;
#77495=CARTESIAN_POINT ( 'NONE',  ( 3.549999999999940314, 2.500000000000000000, 6.941600689897073018 ) ) ;
#77496=CARTESIAN_POINT ( 'NONE',  ( 97.50000000000000000, 0.000000000000000000, 2.000000000000000000 ) ) ;
#77498=EDGE_CURVE ( 'NONE', #80574, #63617, #86068, .T. ) ;
#77499=ADVANCED_FACE ( 'NONE', ( #43612 ), #73498, .T. ) ;
#77500=FACE_OUTER_BOUND ( 'NONE', #50767, .T. ) ;
#77502=ORIENTED_EDGE ( 'NONE', *, *, #58258, .F. ) ;
#77503=DIRECTION ( 'NONE',  ( -4.274815082592931898E-19, -0.9999939076577903929, -0.003490651415223739937 ) ) ;
#77504=AXIS2_PLACEMENT_3D ( 'NONE', #2647, #90383, #70133 ) ;
#77505=AXIS2_PLACEMENT_3D ( 'NONE', #10216, #109035, #91348 ) ;
#77506=VERTEX_POINT ( 'NONE', #45540 ) ;
#77507=CARTESIAN_POINT ( 'NONE',  ( -6.850000000000017408, 2.500000000000000000, -6.841600689897077814 ) ) ;
#77508=EDGE_CURVE ( 'NONE', #114987, #21308, #113202, .T. ) ;
#77510=CARTESIAN_POINT ( 'NONE',  ( 7.049999999999926992, 2.500000000000000000, 2.065063509461097624 ) ) ;
#77511=CARTESIAN_POINT ( 'NONE',  ( -4.150000000000025224, 2.500000000000000000, 2.857883832488649301 ) ) ;
#77512=ORIENTED_EDGE ( 'NONE', *, *, #87571, .T. ) ;
#77513=CARTESIAN_POINT ( 'NONE',  ( -8.350000000000012079, 12.50000000000000000, -1.472243186433550122 ) ) ;
#77514=CARTESIAN_POINT ( 'NONE',  ( -6.450000000000016165, 2.500000000000000000, 6.741600689897071952 ) ) ;
#77515=ORIENTED_EDGE ( 'NONE', *, *, #26084, .T. ) ;
#77516=EDGE_CURVE ( 'NONE', #121748, #28676, #56751, .T. ) ;
#77517=CARTESIAN_POINT ( 'NONE',  ( -9.550000000000006040, 12.50000000000000000, -2.230156782645139391 ) ) ;
#77518=ORIENTED_EDGE ( 'NONE', *, *, #44534, .F. ) ;
#77519=ORIENTED_EDGE ( 'NONE', *, *, #103062, .F. ) ;
#77520=CARTESIAN_POINT ( 'NONE',  ( 5.599999999999933031, 2.500000000000000000, -0.2464101615137783419 ) ) ;
#77521=CARTESIAN_POINT ( 'NONE',  ( -8.100000000000013856, 2.500000000000000000, -3.983716857408426293 ) ) ;
#77523=CARTESIAN_POINT ( 'NONE',  ( -13.74999999999998757, 12.50000000000000000, 1.472243186433549456 ) ) ;
#77524=AXIS2_PLACEMENT_3D ( 'NONE', #52287, #41200, #102661 ) ;
#77525=DIRECTION ( 'NONE',  ( 0.000000000000000000, 0.000000000000000000, 1.000000000000000000 ) ) ;
#77526=CARTESIAN_POINT ( 'NONE',  ( 4.399999999999937295, 2.500000000000000000, 4.576537180435972019 ) ) ;
#77527=VECTOR ( 'NONE', #74524, 1000.000000000000000 ) ;
#77528=EDGE_LOOP ( 'NONE', ( #51385, #43480 ) ) ;
#77529=DIRECTION ( 'NONE',  ( 0.000000000000000000, 0.000000000000000000, 1.000000000000000000 ) ) ;
#77530=LINE ( 'NONE', #14256, #66774 ) ;
#77531=ORIENTED_EDGE ( 'NONE', *, *, #118642, .F. ) ;
#77532=CIRCLE ( 'NONE', #25289, 0.06509327318403741736 ) ;
#77533=DIRECTION ( 'NONE',  ( -0.000000000000000000, 1.000000000000000000, -0.000000000000000000 ) ) ;
#77534=CARTESIAN_POINT ( 'NONE',  ( -13.14999999999999147, 2.500000000000000000, 2.411473670974877415 ) ) ;
#77535=CARTESIAN_POINT ( 'NONE',  ( 11.24999999999991118, 2.500000000000000000, 5.702370205355745014 ) ) ;
#77536=DIRECTION ( 'NONE',  ( 0.000000000000000000, 0.000000000000000000, 1.000000000000000000 ) ) ;
#77537=DIRECTION ( 'NONE',  ( 0.000000000000000000, 0.000000000000000000, 1.000000000000000000 ) ) ;
#77538=ORIENTED_EDGE ( 'NONE', *, *, #83548, .T. ) ;
#77539=ADVANCED_FACE ( 'NONE', ( #126008 ), #79769, .T. ) ;
#77540=FACE_OUTER_BOUND ( 'NONE', #11394, .T. ) ;
#77541=DIRECTION ( 'NONE',  ( 0.000000000000000000, 0.000000000000000000, 1.000000000000000000 ) ) ;
#77542=EDGE_LOOP ( 'NONE', ( #25958, #26235 ) ) ;
#77543=CARTESIAN_POINT ( 'NONE',  ( 9.149999999999920419, 2.500000000000000000, -7.288010851410854585 ) ) ;
#77544=EDGE_CURVE ( 'NONE', #94583, #111170, #23959, .T. ) ;
#77545=EDGE_LOOP ( 'NONE', ( #109459, #117821, #52803, #4573 ) ) ;
#77546=ORIENTED_EDGE ( 'NONE', *, *, #40403, .T. ) ;
#77547=CARTESIAN_POINT ( 'NONE',  ( -14.99999999999998224, 2.500000000000000000, -0.6928203230275519209 ) ) ;
#77549=VECTOR ( 'NONE', #20536, 1000.000000000000000 ) ;
#77550=CIRCLE ( 'NONE', #77644, 0.06509327318403745899 ) ;
#77551=EDGE_LOOP ( 'NONE', ( #64618, #116606, #27008, #47479 ) ) ;
#77552=CARTESIAN_POINT ( 'NONE',  ( -1.650000000000034328, 12.50000000000000000, -2.165063509461101710 ) ) ;
#77553=CARTESIAN_POINT ( 'NONE',  ( -4.150000000000024336, 2.500000000000000000, 1.372243186433545370 ) ) ;
#77554=DIRECTION ( 'NONE',  ( 0.000000000000000000, 0.000000000000000000, -1.000000000000000000 ) ) ;
#77555=VERTEX_POINT ( 'NONE', #74342 ) ;
#77556=CIRCLE ( 'NONE', #113162, 0.1000000000000002554 ) ;
#77557=FACE_BOUND ( 'NONE', #77603, .T. ) ;
#77558=CARTESIAN_POINT ( 'NONE',  ( 3.749999999999944045, 2.500000000000000000, -7.188010851410854052 ) ) ;
#77559=ORIENTED_EDGE ( 'NONE', *, *, #125149, .F. ) ;
#77560=DIRECTION ( 'NONE',  ( 0.000000000000000000, 1.000000000000000000, 0.000000000000000000 ) ) ;
#77561=CARTESIAN_POINT ( 'NONE',  ( -2.500000000000032863, 12.50000000000000000, 5.022947341949748790 ) ) ;
#77562=ORIENTED_EDGE ( 'NONE', *, *, #22355, .T. ) ;
#77563=EDGE_LOOP ( 'NONE', ( #77502, #37609 ) ) ;
#77564=ORIENTED_EDGE ( 'NONE', *, *, #111943, .F. ) ;
#77565=CARTESIAN_POINT ( 'NONE',  ( -4.150000000000025224, 12.50000000000000000, 2.857883832488649301 ) ) ;
#77566=DIRECTION ( 'NONE',  ( 0.000000000000000000, 1.000000000000000000, 0.000000000000000000 ) ) ;
#77567=CARTESIAN_POINT ( 'NONE',  ( -11.04999999999999893, 2.500000000000000000, 1.818653347947321475 ) ) ;
#77568=FACE_BOUND ( 'NONE', #116652, .T. ) ;
#77569=ORIENTED_EDGE ( 'NONE', *, *, #53888, .F. ) ;
#77570=DIRECTION ( 'NONE',  ( -0.000000000000000000, -1.000000000000000000, -0.000000000000000000 ) ) ;
#77571=DIRECTION ( 'NONE',  ( 0.000000000000000000, 1.000000000000000000, 0.000000000000000000 ) ) ;
#77572=ORIENTED_EDGE ( 'NONE', *, *, #120116, .T. ) ;
#77573=EDGE_CURVE ( 'NONE', #102540, #72001, #48465, .T. ) ;
#77574=CIRCLE ( 'NONE', #37880, 0.1000000000000000472 ) ;
#77575=DIRECTION ( 'NONE',  ( -0.000000000000000000, -1.000000000000000000, -0.000000000000000000 ) ) ;
#77576=FACE_OUTER_BOUND ( 'NONE', #85618, .T. ) ;
#77577=CARTESIAN_POINT ( 'NONE',  ( -14.54999999999998472, 2.500000000000000000, 2.265063509461101354 ) ) ;
#77578=CARTESIAN_POINT ( 'NONE',  ( 12.29999999999990656, 2.500000000000000000, -4.676537180435977881 ) ) ;
#77581=ADVANCED_FACE ( 'NONE', ( #93986 ), #114262, .T. ) ;
#77582=AXIS2_PLACEMENT_3D ( 'NONE', #17434, #86168, #66545 ) ;
#77584=ORIENTED_EDGE ( 'NONE', *, *, #28330, .T. ) ;
#77585=EDGE_LOOP ( 'NONE', ( #106814, #122957 ) ) ;
#77586=ORIENTED_EDGE ( 'NONE', *, *, #41212, .F. ) ;
#77587=ORIENTED_EDGE ( 'NONE', *, *, #74212, .F. ) ;
#77588=CARTESIAN_POINT ( 'NONE',  ( 9.799999999999917222, 2.500000000000000000, 0.3464101615137735735 ) ) ;
#77590=DIRECTION ( 'NONE',  ( 0.000000000000000000, 1.000000000000000000, 0.000000000000000000 ) ) ;
#77591=ORIENTED_EDGE ( 'NONE', *, *, #76473, .F. ) ;
#77592=FACE_BOUND ( 'NONE', #70564, .T. ) ;
#77593=EDGE_CURVE ( 'NONE', #104181, #99447, #119462, .T. ) ;
#77594=VECTOR ( 'NONE', #90542, 1000.000000000000000 ) ;
#77595=DIRECTION ( 'NONE',  ( -4.274815082592931898E-19, -0.9999939076577903929, -0.003490651415223739937 ) ) ;
#77596=AXIS2_PLACEMENT_3D ( 'NONE', #82521, #64144, #41949 ) ;
#77597=EDGE_CURVE ( 'NONE', #84209, #1733, #74989, .T. ) ;
#77598=FACE_OUTER_BOUND ( 'NONE', #87562, .T. ) ;
#77600=DIRECTION ( 'NONE',  ( -4.274815082592931898E-19, -0.9999939076577903929, -0.003490651415223739937 ) ) ;
#77601=EDGE_CURVE ( 'NONE', #69877, #66637, #21270, .T. ) ;
#77602=DIRECTION ( 'NONE',  ( 0.000000000000000000, 0.000000000000000000, 1.000000000000000000 ) ) ;
#77603=EDGE_LOOP ( 'NONE', ( #94037, #52189 ) ) ;
#77604=CARTESIAN_POINT ( 'NONE',  ( -5.200000000000020606, 2.500000000000000000, 3.883716857408421319 ) ) ;
#77605=VECTOR ( 'NONE', #9621, 1000.000000000000000 ) ;
#77606=VERTEX_POINT ( 'NONE', #115535 ) ;
#77607=CONICAL_SURFACE ( 'NONE', #21184, 0.1000000000000000472, 0.003490658503988666988 ) ;
#77608=ORIENTED_EDGE ( 'NONE', *, *, #59422, .T. ) ;
#77609=VERTEX_POINT ( 'NONE', #55979 ) ;
#77610=AXIS2_PLACEMENT_3D ( 'NONE', #82877, #31832, #103141 ) ;
#77611=FACE_OUTER_BOUND ( 'NONE', #128851, .T. ) ;
#77612=CARTESIAN_POINT ( 'NONE',  ( -5.650000000000019895, 2.500000000000000000, 6.741600689897071952 ) ) ;
#77613=DIRECTION ( 'NONE',  ( 0.000000000000000000, 0.000000000000000000, 1.000000000000000000 ) ) ;
#77614=ORIENTED_EDGE ( 'NONE', *, *, #90354, .T. ) ;
#77615=CARTESIAN_POINT ( 'NONE',  ( 8.328334241103805269, 2.499999999999999556, -8.539519493613809686 ) ) ;
#77616=CIRCLE ( 'NONE', #21189, 0.1000000000000002554 ) ;
#77617=CARTESIAN_POINT ( 'NONE',  ( 0.1999999999999636513, 12.50000000000000000, -0.3464101615137760715 ) ) ;
#77618=DIRECTION ( 'NONE',  ( 0.000000000000000000, 1.000000000000000000, 0.000000000000000000 ) ) ;
#77619=EDGE_CURVE ( 'NONE', #38510, #115027, #47464, .T. ) ;
#77620=AXIS2_PLACEMENT_3D ( 'NONE', #15274, #55234, #46698 ) ;
#77622=CARTESIAN_POINT ( 'NONE',  ( 13.74999999999989519, 2.500000000000000000, -2.957883832488653830 ) ) ;
#77624=LINE ( 'NONE', #65879, #34931 ) ;
#77625=ORIENTED_EDGE ( 'NONE', *, *, #55666, .T. ) ;
#77626=DIRECTION ( 'NONE',  ( -0.000000000000000000, 1.000000000000000000, -0.000000000000000000 ) ) ;
#77627=VERTEX_POINT ( 'NONE', #118128 ) ;
#77628=ADVANCED_FACE ( 'NONE', ( #38968 ), #108308, .T. ) ;
#77629=EDGE_LOOP ( 'NONE', ( #44094, #22077 ) ) ;
#77630=DIRECTION ( 'NONE',  ( 0.000000000000000000, 0.000000000000000000, 1.000000000000000000 ) ) ;
#77631=PLANE ( 'NONE',  #78086 ) ;
#77632=LINE ( 'NONE', #78314, #16893 ) ;
#77633=ORIENTED_EDGE ( 'NONE', *, *, #61581, .T. ) ;
#77634=ORIENTED_EDGE ( 'NONE', *, *, #23727, .T. ) ;
#77635=ADVANCED_FACE ( 'NONE', ( #88676 ), #19200, .T. ) ;
#77636=CARTESIAN_POINT ( 'NONE',  ( -6.650000000000015454, 2.500000000000000000, 7.188010851410848723 ) ) ;
#77637=DIRECTION ( 'NONE',  ( -0.000000000000000000, 1.000000000000000000, -0.000000000000000000 ) ) ;
#77638=VECTOR ( 'NONE', #17612, 1000.000000000000000 ) ;
#77639=PLANE ( 'NONE',  #14742 ) ;
#77640=ORIENTED_EDGE ( 'NONE', *, *, #74094, .T. ) ;
#77641=ORIENTED_EDGE ( 'NONE', *, *, #114151, .F. ) ;
#77642=CONICAL_SURFACE ( 'NONE', #56701, 0.09999999999999999167, 0.003490658503988666988 ) ;
#77643=EDGE_CURVE ( 'NONE', #45115, #11906, #7524, .T. ) ;
#77644=AXIS2_PLACEMENT_3D ( 'NONE', #58528, #108879, #36944 ) ;
#77645=DIRECTION ( 'NONE',  ( 0.000000000000000000, 0.000000000000000000, 1.000000000000000000 ) ) ;
#77646=EDGE_CURVE ( 'NONE', #98829, #64904, #67203, .T. ) ;
#77647=ADVANCED_FACE ( 'NONE', ( #18637 ), #4516, .T. ) ;
#77648=VERTEX_POINT ( 'NONE', #108938 ) ;
#77649=DIRECTION ( 'NONE',  ( 0.000000000000000000, 0.000000000000000000, 1.000000000000000000 ) ) ;
#77650=AXIS2_PLACEMENT_3D ( 'NONE', #1258, #58895, #88995 ) ;
#77651=CARTESIAN_POINT ( 'NONE',  ( 8.549999999999920774, 2.500000000000000000, 6.148780366869520897 ) ) ;
#77652=VERTEX_POINT ( 'NONE', #19269 ) ;
#77653=CARTESIAN_POINT ( 'NONE',  ( 7.499999999999925393, 12.50000000000000000, -3.637306695894650055 ) ) ;
#77654=AXIS2_PLACEMENT_3D ( 'NONE', #86147, #104515, #54764 ) ;
#77655=ADVANCED_FACE ( 'NONE', ( #127320 ), #111140, .T. ) ;
#77656=DIRECTION ( 'NONE',  ( 0.000000000000000000, 1.000000000000000000, 0.000000000000000000 ) ) ;
#77657=CARTESIAN_POINT ( 'NONE',  ( -10.80000000000000249, 2.500000000000000000, -4.230127018922197557 ) ) ;
#77658=AXIS2_PLACEMENT_3D ( 'NONE', #112910, #63158, #65073 ) ;
#77659=LINE ( 'NONE', #66549, #10340 ) ;
#77660=ORIENTED_EDGE ( 'NONE', *, *, #30915, .T. ) ;
#77661=EDGE_CURVE ( 'NONE', #107053, #49010, #37004, .T. ) ;
#77662=DIRECTION ( 'NONE',  ( 0.000000000000000000, 0.000000000000000000, -1.000000000000000000 ) ) ;
#77663=EDGE_CURVE ( 'NONE', #62516, #104677, #92366, .T. ) ;
#77664=ORIENTED_EDGE ( 'NONE', *, *, #72402, .F. ) ;
#77665=VERTEX_POINT ( 'NONE', #17330 ) ;
#77666=DIRECTION ( 'NONE',  ( -0.000000000000000000, 1.000000000000000000, -0.000000000000000000 ) ) ;
#77667=CARTESIAN_POINT ( 'NONE',  ( -11.64999999999999680, 12.50000000000000000, -6.560283801567336148 ) ) ;
#77668=CARTESIAN_POINT ( 'NONE',  ( -6.249999999999984901, 12.50000000000000000, -2.099970236277064473 ) ) ;
#77669=CARTESIAN_POINT ( 'NONE',  ( -0.4000000000000331624, 12.50000000000000000, -0.6928203230275519209 ) ) ;
#77670=DIRECTION ( 'NONE',  ( -0.000000000000000000, -1.000000000000000000, -0.000000000000000000 ) ) ;
#77671=CARTESIAN_POINT ( 'NONE',  ( -0.6500000000000389910, 2.500000000000000000, -1.818653347947326138 ) ) ;
#77672=DIRECTION ( 'NONE',  ( 0.000000000000000000, 1.000000000000000000, 0.000000000000000000 ) ) ;
#77673=CARTESIAN_POINT ( 'NONE',  ( 9.599999999999914380, 2.500000000000000000, 3.637306695894644726 ) ) ;
#77674=DIRECTION ( 'NONE',  ( -0.000000000000000000, -1.000000000000000000, -0.000000000000000000 ) ) ;
#77675=CARTESIAN_POINT ( 'NONE',  ( 3.749999999999942268, 2.500000000000000000, -5.702370205355749455 ) ) ;
#77676=AXIS2_PLACEMENT_3D ( 'NONE', #75123, #3168, #53556 ) ;
#77677=AXIS2_PLACEMENT_3D ( 'NONE', #5534, #87316, #44842 ) ;
#77678=VERTEX_POINT ( 'NONE', #57285 ) ;
#77679=CARTESIAN_POINT ( 'NONE',  ( 8.349999999999923261, 2.500000000000000000, -6.495190528383302464 ) ) ;
#77680=CARTESIAN_POINT ( 'NONE',  ( 12.09999999999990195, 2.500000000000000000, -0.1000000000000022815 ) ) ;
#77681=DIRECTION ( 'NONE',  ( 0.000000000000000000, 0.000000000000000000, -1.000000000000000000 ) ) ;
#77682=PLANE ( 'NONE',  #6541 ) ;
#77683=CARTESIAN_POINT ( 'NONE',  ( 15.39999999999989200, 2.500000000000000000, -0.7928203230275543412 ) ) ;
#77684=AXIS2_PLACEMENT_3D ( 'NONE', #61487, #82420, #81119 ) ;
#77685=ORIENTED_EDGE ( 'NONE', *, *, #45111, .T. ) ;
#77686=CARTESIAN_POINT ( 'NONE',  ( 14.79999999999989413, 12.50000000000000000, -0.2813168883297408329 ) ) ;
#77687=AXIS2_PLACEMENT_3D ( 'NONE', #42287, #10246, #99279 ) ;
#77688=CARTESIAN_POINT ( 'NONE',  ( -4.600000000000028066, 2.500000000000000000, -5.122947341949753763 ) ) ;
#77689=DIRECTION ( 'NONE',  ( -0.000000000000000000, 1.000000000000000000, -0.000000000000000000 ) ) ;
#77690=EDGE_LOOP ( 'NONE', ( #90599, #102144, #50801, #83884 ) ) ;
#77692=AXIS2_PLACEMENT_3D ( 'NONE', #116190, #54675, #16043 ) ;
#77693=EDGE_LOOP ( 'NONE', ( #4001, #51774 ) ) ;
#77695=EDGE_CURVE ( 'NONE', #28244, #68741, #117390, .T. ) ;
#77696=ORIENTED_EDGE ( 'NONE', *, *, #99648, .F. ) ;
#77697=EDGE_LOOP ( 'NONE', ( #26248, #72719, #71551, #64550 ) ) ;
#77698=ORIENTED_EDGE ( 'NONE', *, *, #24438, .F. ) ;
#77699=AXIS2_PLACEMENT_3D ( 'NONE', #61710, #102270, #41432 ) ;
#77700=CARTESIAN_POINT ( 'NONE',  ( -7.100000000000017408, 12.50000000000000000, -3.637306695894650055 ) ) ;
#77701=AXIS2_PLACEMENT_3D ( 'NONE', #107693, #27187, #57305 ) ;
#77702=FACE_OUTER_BOUND ( 'NONE', #68159, .T. ) ;
#77703=DIRECTION ( 'NONE',  ( 0.000000000000000000, 0.000000000000000000, 1.000000000000000000 ) ) ;
#77704=DIRECTION ( 'NONE',  ( 0.000000000000000000, 0.000000000000000000, -1.000000000000000000 ) ) ;
#77705=ORIENTED_EDGE ( 'NONE', *, *, #62618, .T. ) ;
#77706=AXIS2_PLACEMENT_3D ( 'NONE', #103534, #102245, #32235 ) ;
#77707=CARTESIAN_POINT ( 'NONE',  ( -0.8500000000000386136, 2.500000000000000000, 1.372243186433545370 ) ) ;
#77708=ORIENTED_EDGE ( 'NONE', *, *, #98084, .F. ) ;
#77709=CARTESIAN_POINT ( 'NONE',  ( 65.40459994267393995, -3.824478557797811984, -5.306485876524377865 ) ) ;
#77710=CARTESIAN_POINT ( 'NONE',  ( 15.50772381592132021, -1.500000000000031752, -6.996973294590719483 ) ) ;
#77711=CARTESIAN_POINT ( 'NONE',  ( 3.949999999999941558, 2.500000000000000000, -6.048780366869526581 ) ) ;
#77712=DIRECTION ( 'NONE',  ( 0.000000000000000000, -0.000000000000000000, 1.000000000000000000 ) ) ;
#77713=CARTESIAN_POINT ( 'NONE',  ( 7.099999999999926814, 2.500000000000000000, -0.6928203230275541413 ) ) ;
#77714=VERTEX_POINT ( 'NONE', #129274 ) ;
#77715=ORIENTED_EDGE ( 'NONE', *, *, #109079, .T. ) ;
#77716=ORIENTED_EDGE ( 'NONE', *, *, #48588, .T. ) ;
#77717=ORIENTED_EDGE ( 'NONE', *, *, #87681, .F. ) ;
#77718=DIRECTION ( 'NONE',  ( 0.000000000000000000, 0.000000000000000000, 1.000000000000000000 ) ) ;
#77719=CARTESIAN_POINT ( 'NONE',  ( -3.950000000000024603, 2.500000000000000000, 1.818653347947321475 ) ) ;
#77720=DIRECTION ( 'NONE',  ( -0.000000000000000000, -1.000000000000000000, -0.000000000000000000 ) ) ;
#77721=FACE_BOUND ( 'NONE', #108722, .T. ) ;
#77722=DIRECTION ( 'NONE',  ( 0.000000000000000000, 1.000000000000000000, 0.000000000000000000 ) ) ;
#77723=CARTESIAN_POINT ( 'NONE',  ( -7.050000000000016698, 2.500000000000000000, -6.395190528383301931 ) ) ;
#77724=DIRECTION ( 'NONE',  ( 0.000000000000000000, 1.000000000000000000, 0.000000000000000000 ) ) ;
#77725=DIRECTION ( 'NONE',  ( 0.000000000000000000, 1.000000000000000000, 0.000000000000000000 ) ) ;
#77726=VECTOR ( 'NONE', #73651, 1000.000000000000000 ) ;
#77728=VECTOR ( 'NONE', #90538, 1000.000000000000000 ) ;
#77729=CARTESIAN_POINT ( 'NONE',  ( 7.299999999999927880, 12.50000000000000000, -4.611443907251939756 ) ) ;
#77730=CARTESIAN_POINT ( 'NONE',  ( -2.900000000000029665, 2.500000000000000000, 4.430127018922196847 ) ) ;
#77731=EDGE_CURVE ( 'NONE', #69690, #73131, #127887, .T. ) ;
#77732=DIRECTION ( 'NONE',  ( 0.000000000000000000, 0.000000000000000000, 1.000000000000000000 ) ) ;
#77733=AXIS2_PLACEMENT_3D ( 'NONE', #126438, #3590, #66848 ) ;
#77734=ORIENTED_EDGE ( 'NONE', *, *, #81404, .T. ) ;
#77735=ORIENTED_EDGE ( 'NONE', *, *, #17085, .T. ) ;
#77736=VERTEX_POINT ( 'NONE', #77553 ) ;
#77737=EDGE_LOOP ( 'NONE', ( #116906, #15145, #116198, #53464 ) ) ;
#77739=AXIS2_PLACEMENT_3D ( 'NONE', #101715, #121337, #93821 ) ;
#77741=FACE_OUTER_BOUND ( 'NONE', #60585, .T. ) ;
#77742=FACE_BOUND ( 'NONE', #32265, .T. ) ;
#77743=ADVANCED_FACE ( 'NONE', ( #49414 ), #25551, .T. ) ;
#77744=CONICAL_SURFACE ( 'NONE', #31706, 0.1000000000000002554, 0.003490658503988666988 ) ;
#77745=DIRECTION ( 'NONE',  ( -0.000000000000000000, -1.000000000000000000, -0.000000000000000000 ) ) ;
#77746=EDGE_CURVE ( 'NONE', #41444, #47582, #116831, .T. ) ;
#77747=EDGE_CURVE ( 'NONE', #101182, #55738, #77785, .T. ) ;
#77748=EDGE_LOOP ( 'NONE', ( #87868, #81328, #46778, #80461 ) ) ;
#77749=DIRECTION ( 'NONE',  ( 0.000000000000000000, -0.9999939076577903929, 0.003490651415223739937 ) ) ;
#77750=EDGE_CURVE ( 'NONE', #850, #43290, #42303, .T. ) ;
#77751=CARTESIAN_POINT ( 'NONE',  ( -10.84999999999999964, 2.500000000000000000, 2.957883832488649389 ) ) ;
#77752=EDGE_CURVE ( 'NONE', #72018, #87403, #46829, .T. ) ;
#77753=DIRECTION ( 'NONE',  ( 0.000000000000000000, 0.000000000000000000, 1.000000000000000000 ) ) ;
#77754=ORIENTED_EDGE ( 'NONE', *, *, #60721, .F. ) ;
#77755=DIRECTION ( 'NONE',  ( 0.000000000000000000, 0.000000000000000000, 1.000000000000000000 ) ) ;
#77756=DIRECTION ( 'NONE',  ( 0.000000000000000000, 0.000000000000000000, 1.000000000000000000 ) ) ;
#77757=VERTEX_POINT ( 'NONE', #100430 ) ;
#77758=ORIENTED_EDGE ( 'NONE', *, *, #106885, .F. ) ;
#77759=PLANE ( 'NONE',  #34095 ) ;
#77760=DIRECTION ( 'NONE',  ( 0.000000000000000000, 0.000000000000000000, 1.000000000000000000 ) ) ;
#77761=AXIS2_PLACEMENT_3D ( 'NONE', #46294, #36508, #90079 ) ;
#77762=AXIS2_PLACEMENT_3D ( 'NONE', #117249, #86527, #76074 ) ;
#77763=DIRECTION ( 'NONE',  ( 0.000000000000000000, 1.000000000000000000, 0.000000000000000000 ) ) ;
#77764=DIRECTION ( 'NONE',  ( -0.000000000000000000, -1.000000000000000000, -0.000000000000000000 ) ) ;
#77765=ORIENTED_EDGE ( 'NONE', *, *, #106933, .F. ) ;
#77766=DIRECTION ( 'NONE',  ( 0.000000000000000000, 1.000000000000000000, 0.000000000000000000 ) ) ;
#77767=ORIENTED_EDGE ( 'NONE', *, *, #84572, .F. ) ;
#77768=VERTEX_POINT ( 'NONE', #93670 ) ;
#77769=CARTESIAN_POINT ( 'NONE',  ( -13.09999999999999076, 2.500000000000000000, 3.983716857408420964 ) ) ;
#77770=ORIENTED_EDGE ( 'NONE', *, *, #15603, .T. ) ;
#77771=CARTESIAN_POINT ( 'NONE',  ( -3.100000000000028511, 12.50000000000000000, -4.676537180435977881 ) ) ;
#77772=AXIS2_PLACEMENT_3D ( 'NONE', #25167, #6162, #103743 ) ;
#77773=FACE_BOUND ( 'NONE', #91934, .T. ) ;
#77774=CIRCLE ( 'NONE', #84042, 0.06509327318403745899 ) ;
#77775=EDGE_LOOP ( 'NONE', ( #29910, #12729 ) ) ;
#77776=AXIS2_PLACEMENT_3D ( 'NONE', #43590, #113599, #63857 ) ;
#77777=DIRECTION ( 'NONE',  ( 0.000000000000000000, 1.000000000000000000, 0.000000000000000000 ) ) ;
#77778=EDGE_LOOP ( 'NONE', ( #126538, #68127, #114533, #109959 ) ) ;
#77779=FACE_OUTER_BOUND ( 'NONE', #11609, .T. ) ;
#77780=CARTESIAN_POINT ( 'NONE',  ( -3.350000000000031619, 2.500000000000000000, -5.802370205355749988 ) ) ;
#77781=PLANE ( 'NONE',  #25757 ) ;
#77782=ADVANCED_FACE ( 'NONE', ( #123751 ), #21362, .T. ) ;
#77783=DIRECTION ( 'NONE',  ( -0.000000000000000000, -1.000000000000000000, -0.000000000000000000 ) ) ;
#77784=DIRECTION ( 'NONE',  ( 0.000000000000000000, 1.000000000000000000, 0.000000000000000000 ) ) ;
#77785=CIRCLE ( 'NONE', #109178, 0.06509327318403745899 ) ;
#77786=ORIENTED_EDGE ( 'NONE', *, *, #33326, .T. ) ;
#77787=AXIS2_PLACEMENT_3D ( 'NONE', #23663, #4635, #123156 ) ;
#77788=ORIENTED_EDGE ( 'NONE', *, *, #118023, .F. ) ;
#77789=CARTESIAN_POINT ( 'NONE',  ( -15.59999999999998010, 12.50000000000000000, -0.3464101615137759604 ) ) ;
#77790=FACE_OUTER_BOUND ( 'NONE', #7556, .T. ) ;
#77791=CONICAL_SURFACE ( 'NONE', #66548, 0.1000000000000000056, 0.003490658503988666988 ) ;
#77792=CONICAL_SURFACE ( 'NONE', #21368, 0.09999999999999982514, 0.003490658503988666988 ) ;
#77793=VECTOR ( 'NONE', #42729, 1000.000000000000000 ) ;
#77794=LINE ( 'NONE', #38558, #23007 ) ;
#77795=EDGE_CURVE ( 'NONE', #48968, #27815, #54378, .T. ) ;
#77796=ORIENTED_EDGE ( 'NONE', *, *, #58298, .T. ) ;
#77797=EDGE_LOOP ( 'NONE', ( #16260, #85180 ) ) ;
#77798=ORIENTED_EDGE ( 'NONE', *, *, #64631, .T. ) ;
#77799=ADVANCED_FACE ( 'NONE', ( #110249 ), #48568, .T. ) ;
#77800=DIRECTION ( 'NONE',  ( -0.000000000000000000, 1.000000000000000000, -0.000000000000000000 ) ) ;
#77801=EDGE_CURVE ( 'NONE', #80231, #24379, #119649, .T. ) ;
#77803=FACE_OUTER_BOUND ( 'NONE', #128877, .T. ) ;
#77804=CIRCLE ( 'NONE', #84154, 0.06509327318403745899 ) ;
#77806=DIRECTION ( 'NONE',  ( -4.274815082592931898E-19, -0.9999939076577903929, -0.003490651415223739937 ) ) ;
#77807=LINE ( 'NONE', #10369, #9517 ) ;
#77808=CARTESIAN_POINT ( 'NONE',  ( -10.60000000000000142, 2.500000000000000000, 4.576537180435972019 ) ) ;
#77809=EDGE_CURVE ( 'NONE', #91689, #110749, #10120, .T. ) ;
#77810=EDGE_CURVE ( 'NONE', #98606, #68058, #29775, .T. ) ;
#77812=ADVANCED_FACE ( 'NONE', ( #3355 ), #23415, .T. ) ;
#77813=ORIENTED_EDGE ( 'NONE', *, *, #3738, .T. ) ;
#77814=EDGE_CURVE ( 'NONE', #119917, #129137, #121707, .T. ) ;
#77815=ORIENTED_EDGE ( 'NONE', *, *, #102200, .F. ) ;
#77816=FACE_OUTER_BOUND ( 'NONE', #7447, .T. ) ;
#77817=EDGE_CURVE ( 'NONE', #46788, #79361, #67301, .T. ) ;
#77818=DIRECTION ( 'NONE',  ( 0.000000000000000000, 0.000000000000000000, 1.000000000000000000 ) ) ;
#77819=ORIENTED_EDGE ( 'NONE', *, *, #86045, .F. ) ;
#77820=ORIENTED_EDGE ( 'NONE', *, *, #73274, .T. ) ;
#77822=CARTESIAN_POINT ( 'NONE',  ( 3.299999999999944755, 12.50000000000000000, -4.330127018922201643 ) ) ;
#77823=CARTESIAN_POINT ( 'NONE',  ( -5.450000000000019718, 2.500000000000000000, 2.165063509461097713 ) ) ;
#77825=CARTESIAN_POINT ( 'NONE',  ( 2.899999999999945732, 2.500000000000000000, -2.385244779468109755E-15 ) ) ;
#77826=DIRECTION ( 'NONE',  ( 0.000000000000000000, -0.9999939076577903929, 0.003490651415223739937 ) ) ;
#77827=CARTESIAN_POINT ( 'NONE',  ( -7.500000000000016875, 12.50000000000000000, 0.7579135962115869374 ) ) ;
#77828=AXIS2_PLACEMENT_3D ( 'NONE', #95303, #36398, #16709 ) ;
#77829=DIRECTION ( 'NONE',  ( 0.000000000000000000, 1.000000000000000000, 0.000000000000000000 ) ) ;
#77830=EDGE_LOOP ( 'NONE', ( #76095, #55302, #116761, #128443 ) ) ;
#77831=DIRECTION ( 'NONE',  ( 0.000000000000000000, 1.000000000000000000, 0.000000000000000000 ) ) ;
#77832=VECTOR ( 'NONE', #39972, 1000.000000000000000 ) ;
#77833=CONICAL_SURFACE ( 'NONE', #19240, 0.1000000000000002554, 0.003490658503988666988 ) ;
#77834=DIRECTION ( 'NONE',  ( -0.000000000000000000, 1.000000000000000000, -0.000000000000000000 ) ) ;
#77835=AXIS2_PLACEMENT_3D ( 'NONE', #52393, #91678, #2630 ) ;
#77836=ORIENTED_EDGE ( 'NONE', *, *, #106635, .F. ) ;
#77837=CONICAL_SURFACE ( 'NONE', #8872, 0.1000000000000000056, 0.003490658503988666988 ) ;
#77838=AXIS2_PLACEMENT_3D ( 'NONE', #120473, #51107, #60293 ) ;
#77839=ORIENTED_EDGE ( 'NONE', *, *, #85172, .F. ) ;
#77840=AXIS2_PLACEMENT_3D ( 'NONE', #88582, #47376, #68938 ) ;
#77841=CIRCLE ( 'NONE', #21413, 0.06509327318403745899 ) ;
#77842=ORIENTED_EDGE ( 'NONE', *, *, #79261, .F. ) ;
#77843=VERTEX_POINT ( 'NONE', #21218 ) ;
#77844=FACE_OUTER_BOUND ( 'NONE', #118426, .T. ) ;
#77845=CARTESIAN_POINT ( 'NONE',  ( -7.500000000000015099, 12.50000000000000000, -0.6928203230275541413 ) ) ;
#77846=ORIENTED_EDGE ( 'NONE', *, *, #69202, .F. ) ;
#77847=DIRECTION ( 'NONE',  ( -0.000000000000000000, -1.000000000000000000, -0.000000000000000000 ) ) ;
#77848=CARTESIAN_POINT ( 'NONE',  ( 2.500000000000002220, -2.750000000000000444, -9.999999999999998224 ) ) ;
#77849=CARTESIAN_POINT ( 'NONE',  ( 6.899999999999928413, 2.500000000000000000, -3.883716857408426648 ) ) ;
#77850=CARTESIAN_POINT ( 'NONE',  ( -8.550000000000011369, 12.50000000000000000, 1.753560074763284016 ) ) ;
#77851=ORIENTED_EDGE ( 'NONE', *, *, #55525, .T. ) ;
#77852=LINE ( 'NONE', #7821, #116293 ) ;
#77853=CIRCLE ( 'NONE', #65332, 0.1000000000000002554 ) ;
#77854=CARTESIAN_POINT ( 'NONE',  ( -0.4000000000000401013, 12.50000000000000000, -3.637306695894650055 ) ) ;
#77855=ORIENTED_EDGE ( 'NONE', *, *, #61610, .T. ) ;
#77856=ADVANCED_FACE ( 'NONE', ( #10729 ), #19296, .T. ) ;
#77857=ORIENTED_EDGE ( 'NONE', *, *, #72073, .T. ) ;
#77858=ORIENTED_EDGE ( 'NONE', *, *, #18339, .F. ) ;
#77859=CARTESIAN_POINT ( 'NONE',  ( -3.550000000000028688, 12.50000000000000000, 6.841600689897072485 ) ) ;
#77860=CIRCLE ( 'NONE', #33967, 0.06509327318403745899 ) ;
#77861=DIRECTION ( 'NONE',  ( 0.000000000000000000, 0.000000000000000000, -1.000000000000000000 ) ) ;
#77862=CIRCLE ( 'NONE', #591, 0.06509327318403745899 ) ;
#77863=ORIENTED_EDGE ( 'NONE', *, *, #126983, .T. ) ;
#77864=DIRECTION ( 'NONE',  ( -0.000000000000000000, 1.000000000000000000, -0.000000000000000000 ) ) ;
#77865=CARTESIAN_POINT ( 'NONE',  ( 7.699999999999925571, 2.500000000000000000, -4.676537180435978769 ) ) ;
#77866=ADVANCED_FACE ( 'NONE', ( #34768 ), #88241, .T. ) ;
#77867=DIRECTION ( 'NONE',  ( 0.000000000000000000, 0.000000000000000000, 1.000000000000000000 ) ) ;
#77868=FACE_OUTER_BOUND ( 'NONE', #41943, .T. ) ;
#77870=AXIS2_PLACEMENT_3D ( 'NONE', #111415, #169, #29654 ) ;
#77871=VERTEX_POINT ( 'NONE', #276 ) ;
#77872=CARTESIAN_POINT ( 'NONE',  ( 9.399999999999918643, 2.500000000000000000, 0.3464101615137736845 ) ) ;
#77873=AXIS2_PLACEMENT_3D ( 'NONE', #24419, #32338, #114725 ) ;
#77874=ORIENTED_EDGE ( 'NONE', *, *, #100470, .T. ) ;
#77875=ORIENTED_EDGE ( 'NONE', *, *, #4436, .T. ) ;
#77876=DIRECTION ( 'NONE',  ( -0.000000000000000000, -1.000000000000000000, -0.000000000000000000 ) ) ;
#77877=DIRECTION ( 'NONE',  ( 0.000000000000000000, 0.000000000000000000, 1.000000000000000000 ) ) ;
#77878=FACE_BOUND ( 'NONE', #5287, .T. ) ;
#77879=DIRECTION ( 'NONE',  ( 0.000000000000000000, 1.000000000000000000, 0.000000000000000000 ) ) ;
#77880=CONICAL_SURFACE ( 'NONE', #115521, 0.09999999999999999167, 0.003490658503988666988 ) ;
#77881=DIRECTION ( 'NONE',  ( 0.000000000000000000, 0.000000000000000000, -1.000000000000000000 ) ) ;
#77882=CARTESIAN_POINT ( 'NONE',  ( 4.149999999999936406, 12.50000000000000000, 6.495190528383297135 ) ) ;
#77883=CIRCLE ( 'NONE', #73678, 0.1000000000000002554 ) ;
#77884=AXIS2_PLACEMENT_3D ( 'NONE', #676, #23536, #62202 ) ;
#77885=EDGE_LOOP ( 'NONE', ( #14764, #8028, #49055, #127140 ) ) ;
#77887=CARTESIAN_POINT ( 'NONE',  ( -7.100000000000018296, 2.500000000000000000, -2.385244779468109755E-15 ) ) ;
#77888=DIRECTION ( 'NONE',  ( 0.000000000000000000, -0.9999939076577903929, 0.003490651415223739937 ) ) ;
#77889=AXIS2_PLACEMENT_3D ( 'NONE', #115082, #36569, #104632 ) ;
#77890=FACE_OUTER_BOUND ( 'NONE', #124926, .T. ) ;
#77892=CARTESIAN_POINT ( 'NONE',  ( -1.450000000000036371, 12.50000000000000000, 6.841600689897072485 ) ) ;
#77894=FACE_OUTER_BOUND ( 'NONE', #32936, .T. ) ;
#77895=AXIS2_PLACEMENT_3D ( 'NONE', #110455, #1778, #120289 ) ;
#77896=ORIENTED_EDGE ( 'NONE', *, *, #98847, .F. ) ;
#77897=ORIENTED_EDGE ( 'NONE', *, *, #6979, .T. ) ;
#77898=FACE_OUTER_BOUND ( 'NONE', #48851, .T. ) ;
#77899=CARTESIAN_POINT ( 'NONE',  ( -0.6500000000000389910, 2.500000000000000000, -6.248780366869526759 ) ) ;
#77900=FACE_BOUND ( 'NONE', #117534, .T. ) ;
#77901=EDGE_CURVE ( 'NONE', #113533, #97281, #6665, .T. ) ;
#77902=CARTESIAN_POINT ( 'NONE',  ( -0.8500000000000382805, 2.500000000000000000, -1.472243186433550122 ) ) ;
#77903=ORIENTED_EDGE ( 'NONE', *, *, #92153, .T. ) ;
#77904=LINE ( 'NONE', #87080, #56940 ) ;
#77905=EDGE_CURVE ( 'NONE', #73152, #19309, #80804, .T. ) ;
#77906=EDGE_LOOP ( 'NONE', ( #109034, #63246 ) ) ;
#77907=ADVANCED_FACE ( 'NONE', ( #113955 ), #33475, .T. ) ;
#77908=EDGE_LOOP ( 'NONE', ( #122078, #24235 ) ) ;
#77909=CARTESIAN_POINT ( 'NONE',  ( -8.950000000000006395, 2.500000000000000000, 6.741600689897071952 ) ) ;
#77910=AXIS2_PLACEMENT_3D ( 'NONE', #90390, #729, #40694 ) ;
#77911=ADVANCED_FACE ( 'NONE', ( #53741 ), #38101, .T. ) ;
#77912=EDGE_CURVE ( 'NONE', #88678, #119766, #6756, .T. ) ;
#77914=EDGE_CURVE ( 'NONE', #24096, #19955, #63133, .T. ) ;
#77915=ORIENTED_EDGE ( 'NONE', *, *, #28112, .F. ) ;
#77916=CARTESIAN_POINT ( 'NONE',  ( -8.100000000000010303, 2.500000000000000000, 3.983716857408420964 ) ) ;
#77917=CARTESIAN_POINT ( 'NONE',  ( -5.600000000000020073, 2.500000000000000000, 4.083716857408421497 ) ) ;
#77918=AXIS2_PLACEMENT_3D ( 'NONE', #73555, #31719, #33026 ) ;
#77919=AXIS2_PLACEMENT_3D ( 'NONE', #2594, #81807, #121733 ) ;
#77920=CONICAL_SURFACE ( 'NONE', #13061, 0.1000000000000002554, 0.003490658503988666988 ) ;
#77921=PLANE ( 'NONE',  #27726 ) ;
#77922=DIRECTION ( 'NONE',  ( 0.000000000000000000, 0.000000000000000000, 1.000000000000000000 ) ) ;
#77924=ADVANCED_FACE ( 'NONE', ( #65487 ), #84052, .T. ) ;
#77925=CIRCLE ( 'NONE', #86331, 0.1000000000000002554 ) ;
#77926=EDGE_CURVE ( 'NONE', #61216, #69514, #36042, .T. ) ;
#77927=AXIS2_PLACEMENT_3D ( 'NONE', #108443, #60656, #38445 ) ;
#77928=EDGE_LOOP ( 'NONE', ( #38286, #15060 ) ) ;
#77929=CONICAL_SURFACE ( 'NONE', #90436, 0.1000000000000002554, 0.003490658503988666988 ) ;
#77930=DIRECTION ( 'NONE',  ( -0.000000000000000000, -1.000000000000000000, -0.000000000000000000 ) ) ;
#77931=DIRECTION ( 'NONE',  ( 0.000000000000000000, 0.000000000000000000, 1.000000000000000000 ) ) ;
#77932=LINE ( 'NONE', #109328, #55534 ) ;
#77933=AXIS2_PLACEMENT_3D ( 'NONE', #56845, #103572, #83288 ) ;
#77934=DIRECTION ( 'NONE',  ( 0.000000000000000000, 0.000000000000000000, 1.000000000000000000 ) ) ;
#77935=AXIS2_PLACEMENT_3D ( 'NONE', #6016, #83934, #85238 ) ;
#77936=EDGE_LOOP ( 'NONE', ( #125794, #98299, #81230, #29057 ) ) ;
#77937=DIRECTION ( 'NONE',  ( 0.000000000000000000, 1.000000000000000000, 0.000000000000000000 ) ) ;
#77938=ORIENTED_EDGE ( 'NONE', *, *, #99977, .F. ) ;
#77939=FACE_OUTER_BOUND ( 'NONE', #86268, .T. ) ;
#77940=AXIS2_PLACEMENT_3D ( 'NONE', #129396, #97326, #99911 ) ;
#77941=ORIENTED_EDGE ( 'NONE', *, *, #120335, .F. ) ;
#77942=DIRECTION ( 'NONE',  ( 0.000000000000000000, -0.000000000000000000, 1.000000000000000000 ) ) ;
#77943=CARTESIAN_POINT ( 'NONE',  ( 87.49999999999995737, -5.708722954879577927, -4.899943752027913213 ) ) ;
#77945=DIRECTION ( 'NONE',  ( -4.274815082592931898E-19, -0.9999939076577903929, -0.003490651415223739937 ) ) ;
#77946=ORIENTED_EDGE ( 'NONE', *, *, #97843, .T. ) ;
#77947=CARTESIAN_POINT ( 'NONE',  ( 8.749999999999957367, 2.500000000000000000, -6.595190528383302109 ) ) ;
#77948=CARTESIAN_POINT ( 'NONE',  ( -10.80000000000000071, 2.500000000000000000, 4.330127018922196314 ) ) ;
#77949=CARTESIAN_POINT ( 'NONE',  ( 4.349999999999938360, 2.500000000000000000, 1.818653347947321475 ) ) ;
#77950=DIRECTION ( 'NONE',  ( -4.274815082592931898E-19, -0.9999939076577903929, -0.003490651415223739937 ) ) ;
#77952=CONICAL_SURFACE ( 'NONE', #94675, 0.1000000000000000472, 0.003490658503988666988 ) ;
#77953=EDGE_LOOP ( 'NONE', ( #6733, #84399, #121483, #23154 ) ) ;
#77954=EDGE_LOOP ( 'NONE', ( #49148, #26107, #117588, #47379 ) ) ;
#77955=DIRECTION ( 'NONE',  ( 0.000000000000000000, 0.000000000000000000, 1.000000000000000000 ) ) ;
#77956=VERTEX_POINT ( 'NONE', #36699 ) ;
#77957=DIRECTION ( 'NONE',  ( -0.000000000000000000, 1.000000000000000000, -0.000000000000000000 ) ) ;
#77958=VERTEX_POINT ( 'NONE', #87059 ) ;
#77959=EDGE_LOOP ( 'NONE', ( #98342, #92852, #37183, #16097 ) ) ;
#77960=ORIENTED_EDGE ( 'NONE', *, *, #78530, .F. ) ;
#77961=FACE_OUTER_BOUND ( 'NONE', #67008, .T. ) ;
#77962=AXIS2_PLACEMENT_3D ( 'NONE', #69997, #109924, #587 ) ;
#77963=CIRCLE ( 'NONE', #113469, 0.06509327318403743123 ) ;
#77964=CARTESIAN_POINT ( 'NONE',  ( -10.00000000000000533, 2.500000000000000000, 5.022947341949748790 ) ) ;
#77965=CONICAL_SURFACE ( 'NONE', #34151, 0.1000000000000002554, 0.003490658503988666988 ) ;
#77966=CARTESIAN_POINT ( 'NONE',  ( 2.949999999999943334, 2.500000000000000000, 6.495190528383297135 ) ) ;
#77968=DIRECTION ( 'NONE',  ( 0.000000000000000000, 0.000000000000000000, 1.000000000000000000 ) ) ;
#77969=LINE ( 'NONE', #117886, #39717 ) ;
#77970=FACE_OUTER_BOUND ( 'NONE', #71446, .T. ) ;
#77971=DIRECTION ( 'NONE',  ( 0.000000000000000000, 0.000000000000000000, 1.000000000000000000 ) ) ;
#77972=ADVANCED_FACE ( 'NONE', ( #94968 ), #56939, .T. ) ;
#77973=VECTOR ( 'NONE', #128310, 1000.000000000000000 ) ;
#77974=CIRCLE ( 'NONE', #121786, 0.09999999999999982514 ) ;
#77975=DIRECTION ( 'NONE',  ( -0.000000000000000000, 1.000000000000000000, -0.000000000000000000 ) ) ;
#77976=ORIENTED_EDGE ( 'NONE', *, *, #119181, .F. ) ;
#77977=EDGE_CURVE ( 'NONE', #30581, #1004, #105429, .T. ) ;
#77978=CONICAL_SURFACE ( 'NONE', #63307, 0.09999999999999982514, 0.003490658503988666988 ) ;
#77979=EDGE_LOOP ( 'NONE', ( #123505, #73608, #99048, #57671 ) ) ;
#77980=ORIENTED_EDGE ( 'NONE', *, *, #42088, .T. ) ;
#77981=CONICAL_SURFACE ( 'NONE', #36134, 0.1000000000000002554, 0.003490658503988666988 ) ;
#77982=EDGE_LOOP ( 'NONE', ( #82661, #10982 ) ) ;
#77983=EDGE_CURVE ( 'NONE', #11927, #42980, #96563, .T. ) ;
#77984=DIRECTION ( 'NONE',  ( -0.000000000000000000, 1.000000000000000000, -0.000000000000000000 ) ) ;
#77985=ORIENTED_EDGE ( 'NONE', *, *, #96975, .T. ) ;
#77986=ORIENTED_EDGE ( 'NONE', *, *, #56811, .T. ) ;
#77987=CIRCLE ( 'NONE', #38285, 0.1000000000000000472 ) ;
#77988=EDGE_CURVE ( 'NONE', #37050, #40625, #10871, .T. ) ;
#77989=CARTESIAN_POINT ( 'NONE',  ( 7.949999999999922018, 2.500000000000000000, -2.165063509461101710 ) ) ;
#77990=CARTESIAN_POINT ( 'NONE',  ( -2.500000000000032419, 12.50000000000000000, -3.572213422710612374 ) ) ;
#77991=DIRECTION ( 'NONE',  ( 0.000000000000000000, 0.000000000000000000, 1.000000000000000000 ) ) ;
#77992=CIRCLE ( 'NONE', #38290, 0.09999999999999982514 ) ;
#77993=DIRECTION ( 'NONE',  ( -0.000000000000000000, 1.000000000000000000, -0.000000000000000000 ) ) ;
#77994=DIRECTION ( 'NONE',  ( 0.000000000000000000, 0.000000000000000000, 1.000000000000000000 ) ) ;
#77995=EDGE_LOOP ( 'NONE', ( #1634, #63471, #67792, #42929 ) ) ;
#77996=AXIS2_PLACEMENT_3D ( 'NONE', #110436, #1130, #120275 ) ;
#77997=DIRECTION ( 'NONE',  ( -0.000000000000000000, -1.000000000000000000, -0.000000000000000000 ) ) ;
#77998=VERTEX_POINT ( 'NONE', #45222 ) ;
#77999=DIRECTION ( 'NONE',  ( 0.000000000000000000, 0.000000000000000000, -1.000000000000000000 ) ) ;
#78000=ORIENTED_EDGE ( 'NONE', *, *, #127310, .T. ) ;
#78002=CARTESIAN_POINT ( 'NONE',  ( -12.09999999999999432, 2.500000000000000000, 3.737306695894644371 ) ) ;
#78004=ADVANCED_FACE ( 'NONE', ( #115883 ), #65267, .T. ) ;
#78005=EDGE_LOOP ( 'NONE', ( #26334, #107377, #121590, #40068 ) ) ;
#78006=CARTESIAN_POINT ( 'NONE',  ( -8.350000000000013856, 2.500000000000000000, -7.188010851410848723 ) ) ;
#78007=CARTESIAN_POINT ( 'NONE',  ( -12.94999999999999218, 2.500000000000000000, 2.165063509461101265 ) ) ;
#78008=DIRECTION ( 'NONE',  ( 0.000000000000000000, -0.9999939076577903929, 0.003490651415223739937 ) ) ;
#78009=DIRECTION ( 'NONE',  ( 0.000000000000000000, -0.9999939076577903929, 0.003490651415223739937 ) ) ;
#78010=CARTESIAN_POINT ( 'NONE',  ( -10.65000000000000391, 12.50000000000000000, -6.776507416713037912 ) ) ;
#78011=ORIENTED_EDGE ( 'NONE', *, *, #127328, .F. ) ;
#78012=LINE ( 'NONE', #48564, #116782 ) ;
#78013=DIRECTION ( 'NONE',  ( -0.000000000000000000, -1.000000000000000000, -0.000000000000000000 ) ) ;
#78014=CONICAL_SURFACE ( 'NONE', #88467, 0.1000000000000002554, 0.003490658503988666988 ) ;
#78015=DIRECTION ( 'NONE',  ( 0.000000000000000000, 0.000000000000000000, 1.000000000000000000 ) ) ;
#78016=DIRECTION ( 'NONE',  ( -0.000000000000000000, -1.000000000000000000, -0.000000000000000000 ) ) ;
#78017=LINE ( 'NONE', #40039, #100042 ) ;
#78018=ORIENTED_EDGE ( 'NONE', *, *, #98019, .T. ) ;
#78019=CIRCLE ( 'NONE', #98953, 0.06509327318403745899 ) ;
#78020=EDGE_CURVE ( 'NONE', #126618, #117214, #36041, .T. ) ;
#78021=AXIS2_PLACEMENT_3D ( 'NONE', #12696, #93224, #82105 ) ;
#78022=ORIENTED_EDGE ( 'NONE', *, *, #18503, .T. ) ;
#78023=CIRCLE ( 'NONE', #71769, 0.1000000000000000472 ) ;
#78024=CIRCLE ( 'NONE', #71770, 0.1000000000000002554 ) ;
#78025=DIRECTION ( 'NONE',  ( 0.000000000000000000, 1.000000000000000000, 0.000000000000000000 ) ) ;
#78026=VERTEX_POINT ( 'NONE', #85127 ) ;
#78027=CARTESIAN_POINT ( 'NONE',  ( 9.599999999999914380, 12.50000000000000000, -4.395220292106239768 ) ) ;
#78029=CIRCLE ( 'NONE', #75874, 0.06509327318403745899 ) ;
#78030=AXIS2_PLACEMENT_3D ( 'NONE', #78139, #38883, #30338 ) ;
#78031=CIRCLE ( 'NONE', #82244, 0.09999999999999982514 ) ;
#78032=AXIS2_PLACEMENT_3D ( 'NONE', #21455, #41766, #81662 ) ;
#78033=CIRCLE ( 'NONE', #103167, 0.06509327318403745899 ) ;
#78036=DIRECTION ( 'NONE',  ( -4.274815082592931898E-19, -0.9999939076577903929, -0.003490651415223739937 ) ) ;
#78037=EDGE_CURVE ( 'NONE', #17665, #34687, #96879, .T. ) ;
#78038=DIRECTION ( 'NONE',  ( -0.000000000000000000, -1.000000000000000000, -0.000000000000000000 ) ) ;
#78039=PLANE ( 'NONE',  #1649 ) ;
#78040=ORIENTED_EDGE ( 'NONE', *, *, #83289, .F. ) ;
#78041=CIRCLE ( 'NONE', #71784, 0.09999999999999982514 ) ;
#78042=DIRECTION ( 'NONE',  ( 0.000000000000000000, 0.000000000000000000, -1.000000000000000000 ) ) ;
#78043=DIRECTION ( 'NONE',  ( 0.000000000000000000, -0.000000000000000000, 1.000000000000000000 ) ) ;
#78044=EDGE_LOOP ( 'NONE', ( #24712, #29050, #101978, #62291 ) ) ;
#78045=CARTESIAN_POINT ( 'NONE',  ( -5.400000000000019895, 2.500000000000000000, 3.637306695894644726 ) ) ;
#78046=DIRECTION ( 'NONE',  ( 0.000000000000000000, 1.000000000000000000, 0.000000000000000000 ) ) ;
#78047=DIRECTION ( 'NONE',  ( 0.000000000000000000, 0.000000000000000000, -1.000000000000000000 ) ) ;
#78048=AXIS2_PLACEMENT_3D ( 'NONE', #17840, #87856, #78053 ) ;
#78049=EDGE_LOOP ( 'NONE', ( #83332, #107779, #77538, #14759 ) ) ;
#78051=EDGE_LOOP ( 'NONE', ( #82753, #119935 ) ) ;
#78052=DIRECTION ( 'NONE',  ( 0.000000000000000000, 1.000000000000000000, 0.000000000000000000 ) ) ;
#78053=DIRECTION ( 'NONE',  ( 0.000000000000000000, 0.000000000000000000, 1.000000000000000000 ) ) ;
#78054=CARTESIAN_POINT ( 'NONE',  ( -0.4000000000000396572, 2.500000000000000000, 3.537306695894645081 ) ) ;
#78055=AXIS2_PLACEMENT_3D ( 'NONE', #5734, #93499, #3822 ) ;
#78056=ORIENTED_EDGE ( 'NONE', *, *, #44596, .T. ) ;
#78057=VECTOR ( 'NONE', #76158, 1000.000000000000000 ) ;
#78058=CIRCLE ( 'NONE', #21633, 0.09999999999999982514 ) ;
#78059=DIRECTION ( 'NONE',  ( 0.000000000000000000, 0.000000000000000000, 1.000000000000000000 ) ) ;
#78060=ADVANCED_FACE ( 'NONE', ( #127005 ), #105062, .T. ) ;
#78061=DIRECTION ( 'NONE',  ( 0.000000000000000000, -0.9999939076577903929, 0.003490651415223739937 ) ) ;
#78062=EDGE_LOOP ( 'NONE', ( #93824, #93288 ) ) ;
#78063=DIRECTION ( 'NONE',  ( 0.000000000000000000, 0.000000000000000000, 1.000000000000000000 ) ) ;
#78064=EDGE_LOOP ( 'NONE', ( #28534, #67799 ) ) ;
#78065=VECTOR ( 'NONE', #36484, 1000.000000000000000 ) ;
#78066=FACE_OUTER_BOUND ( 'NONE', #51499, .T. ) ;
#78067=CIRCLE ( 'NONE', #109462, 0.09999999999999982514 ) ;
#78068=ADVANCED_FACE ( 'NONE', ( #55673 ), #127637, .T. ) ;
#78069=AXIS2_PLACEMENT_3D ( 'NONE', #64182, #2036, #92345 ) ;
#78070=VERTEX_POINT ( 'NONE', #37968 ) ;
#78071=DIRECTION ( 'NONE',  ( 0.000000000000000000, 0.000000000000000000, 1.000000000000000000 ) ) ;
#78072=CARTESIAN_POINT ( 'NONE',  ( -14.34999999999998543, 12.50000000000000000, -1.818653347947323695 ) ) ;
#78073=EDGE_CURVE ( 'NONE', #71153, #123556, #26224, .T. ) ;
#78074=ORIENTED_EDGE ( 'NONE', *, *, #6816, .F. ) ;
#78075=EDGE_CURVE ( 'NONE', #46687, #129191, #29874, .T. ) ;
#78076=ORIENTED_EDGE ( 'NONE', *, *, #24118, .T. ) ;
#78077=ADVANCED_FACE ( 'NONE', ( #64841 ), #77880, .T. ) ;
#78078=CIRCLE ( 'NONE', #57144, 0.1000000000000002554 ) ;
#78079=EDGE_CURVE ( 'NONE', #22492, #55110, #23606, .T. ) ;
#78080=FACE_OUTER_BOUND ( 'NONE', #115164, .T. ) ;
#78081=CARTESIAN_POINT ( 'NONE',  ( 9.349999999999916156, 2.500000000000000000, 6.148780366869520009 ) ) ;
#78082=VERTEX_POINT ( 'NONE', #60838 ) ;
#78084=CARTESIAN_POINT ( 'NONE',  ( -11.25000000000000178, 12.50000000000000000, -5.802370205355746435 ) ) ;
#78085=CIRCLE ( 'NONE', #42505, 0.06509327318403745899 ) ;
#78086=AXIS2_PLACEMENT_3D ( 'NONE', #88079, #58660, #58019 ) ;
#78087=EDGE_CURVE ( 'NONE', #93720, #109560, #109284, .T. ) ;
#78088=CARTESIAN_POINT ( 'NONE',  ( -9.150000000000009237, 2.500000000000000000, -2.857883832488653741 ) ) ;
#78089=DIRECTION ( 'NONE',  ( 0.000000000000000000, 0.000000000000000000, 1.000000000000000000 ) ) ;
#78090=EDGE_CURVE ( 'NONE', #31018, #46687, #89655, .T. ) ;
#78091=FACE_OUTER_BOUND ( 'NONE', #20475, .T. ) ;
#78092=CIRCLE ( 'NONE', #63423, 0.1000000000000000056 ) ;
#78093=DIRECTION ( 'NONE',  ( 0.000000000000000000, 0.000000000000000000, -1.000000000000000000 ) ) ;
#78094=EDGE_CURVE ( 'NONE', #40852, #73230, #86281, .T. ) ;
#78095=AXIS2_PLACEMENT_3D ( 'NONE', #129139, #116700, #108168 ) ;
#78096=EDGE_CURVE ( 'NONE', #77488, #117879, #8923, .T. ) ;
#78097=EDGE_CURVE ( 'NONE', #48532, #92622, #69351, .T. ) ;
#78098=ORIENTED_EDGE ( 'NONE', *, *, #80811, .F. ) ;
#78099=ORIENTED_EDGE ( 'NONE', *, *, #82395, .T. ) ;
#78100=ORIENTED_EDGE ( 'NONE', *, *, #38941, .T. ) ;
#78101=ORIENTED_EDGE ( 'NONE', *, *, #82081, .T. ) ;
#78102=CARTESIAN_POINT ( 'NONE',  ( -9.550000000000007816, 2.500000000000000000, -6.395190528383296602 ) ) ;
#78103=DIRECTION ( 'NONE',  ( 0.000000000000000000, -0.9999939076577903929, 0.003490651415223739937 ) ) ;
#78104=CARTESIAN_POINT ( 'NONE',  ( 12.29999999999990656, 2.500000000000000000, -4.576537180435977348 ) ) ;
#78105=ORIENTED_EDGE ( 'NONE', *, *, #2127, .F. ) ;
#78106=FACE_BOUND ( 'NONE', #122000, .T. ) ;
#78107=ORIENTED_EDGE ( 'NONE', *, *, #125569, .F. ) ;
#78108=EDGE_CURVE ( 'NONE', #118058, #100004, #54899, .T. ) ;
#78109=FACE_OUTER_BOUND ( 'NONE', #28744, .T. ) ;
#78110=DIRECTION ( 'NONE',  ( 0.000000000000000000, -0.9999939076577903929, 0.003490651415223739937 ) ) ;
#78112=DIRECTION ( 'NONE',  ( 0.000000000000000000, 0.000000000000000000, 1.000000000000000000 ) ) ;
#78113=FACE_OUTER_BOUND ( 'NONE', #44306, .T. ) ;
#78114=LINE ( 'NONE', #8695, #106177 ) ;
#78115=DIRECTION ( 'NONE',  ( 0.000000000000000000, 0.000000000000000000, 1.000000000000000000 ) ) ;
#78116=CARTESIAN_POINT ( 'NONE',  ( -1.450000000000035039, 2.500000000000000000, -6.841600689897077814 ) ) ;
#78117=VECTOR ( 'NONE', #92147, 1000.000000000000000 ) ;
#78118=CONICAL_SURFACE ( 'NONE', #97068, 0.1000000000000002554, 0.003490658503988666988 ) ;
#78119=DIRECTION ( 'NONE',  ( 0.000000000000000000, 0.000000000000000000, 1.000000000000000000 ) ) ;
#78120=CARTESIAN_POINT ( 'NONE',  ( -0.8500000000000382805, 12.50000000000000000, -7.188010851410854052 ) ) ;
#78121=CIRCLE ( 'NONE', #36364, 0.06509327318403745899 ) ;
#78122=CIRCLE ( 'NONE', #48889, 10.00000000000000000 ) ;
#78123=ORIENTED_EDGE ( 'NONE', *, *, #120346, .F. ) ;
#78124=ORIENTED_EDGE ( 'NONE', *, *, #120476, .T. ) ;
#78125=EDGE_LOOP ( 'NONE', ( #40283, #89564 ) ) ;
#78126=AXIS2_PLACEMENT_3D ( 'NONE', #120911, #10318, #474 ) ;
#78127=ORIENTED_EDGE ( 'NONE', *, *, #67369, .T. ) ;
#78128=CARTESIAN_POINT ( 'NONE',  ( -3.550000000000027800, 12.50000000000000000, 6.148780366869520009 ) ) ;
#78129=CONICAL_SURFACE ( 'NONE', #9160, 0.09999999999999982514, 0.003490658503988666988 ) ;
#78130=CIRCLE ( 'NONE', #21693, 0.09999999999999999167 ) ;
#78131=LINE ( 'NONE', #67643, #10918 ) ;
#78132=EDGE_LOOP ( 'NONE', ( #50263, #82740 ) ) ;
#78133=ORIENTED_EDGE ( 'NONE', *, *, #90693, .F. ) ;
#78134=ORIENTED_EDGE ( 'NONE', *, *, #764, .F. ) ;
#78135=CARTESIAN_POINT ( 'NONE',  ( -4.400000000000028777, 12.50000000000000000, -4.741630453620016006 ) ) ;
#78136=CIRCLE ( 'NONE', #55041, 0.1000000000000002554 ) ;
#78137=CIRCLE ( 'NONE', #88484, 0.09999999999999982514 ) ;
#78138=CONICAL_SURFACE ( 'NONE', #128316, 0.1000000000000002554, 0.003490658503988666988 ) ;
#78139=CARTESIAN_POINT ( 'NONE',  ( 12.94999999999990337, 12.50000000000000000, 2.165063509461097713 ) ) ;
#78140=CARTESIAN_POINT ( 'NONE',  ( -1.250000000000036193, 12.50000000000000000, 1.407149913249508000 ) ) ;
#78141=CARTESIAN_POINT ( 'NONE',  ( -2.500000000000032863, 2.500000000000000000, 4.922947341949748257 ) ) ;
#78142=CARTESIAN_POINT ( 'NONE',  ( -0.6000000000000323963, 2.500000000000000000, 0.4464101615137759382 ) ) ;
#78143=DIRECTION ( 'NONE',  ( 0.000000000000000000, 1.000000000000000000, 0.000000000000000000 ) ) ;
#78144=CIRCLE ( 'NONE', #11216, 0.1000000000000000472 ) ;
#78145=CARTESIAN_POINT ( 'NONE',  ( -7.100000000000017408, 2.500000000000000000, -0.6928203230275542523 ) ) ;
#78146=ORIENTED_EDGE ( 'NONE', *, *, #76831, .F. ) ;
#78147=DIRECTION ( 'NONE',  ( -0.000000000000000000, -1.000000000000000000, -0.000000000000000000 ) ) ;
#78148=ORIENTED_EDGE ( 'NONE', *, *, #22996, .T. ) ;
#78149=ADVANCED_FACE ( 'NONE', ( #128955 ), #119111, .T. ) ;
#78150=VERTEX_POINT ( 'NONE', #39920 ) ;
#78151=VERTEX_POINT ( 'NONE', #70652 ) ;
#78153=DIRECTION ( 'NONE',  ( 0.000000000000000000, 1.000000000000000000, 0.000000000000000000 ) ) ;
#78154=EDGE_LOOP ( 'NONE', ( #39662, #11210 ) ) ;
#78155=ORIENTED_EDGE ( 'NONE', *, *, #121136, .T. ) ;
#78156=AXIS2_PLACEMENT_3D ( 'NONE', #55679, #87709, #96888 ) ;
#78157=CARTESIAN_POINT ( 'NONE',  ( 9.599999999999914380, 12.50000000000000000, -5.022947341949754119 ) ) ;
#78158=EDGE_CURVE ( 'NONE', #79022, #107927, #82097, .T. ) ;
#78159=CARTESIAN_POINT ( 'NONE',  ( 11.24999999999994493, 2.500000000000000000, -2.265063509461101798 ) ) ;
#78160=DIRECTION ( 'NONE',  ( -0.000000000000000000, 1.000000000000000000, -0.000000000000000000 ) ) ;
#78161=CARTESIAN_POINT ( 'NONE',  ( -0.6500000000000389910, 12.50000000000000000, -6.083687093685488989 ) ) ;
#78162=DIRECTION ( 'NONE',  ( -0.000000000000000000, -1.000000000000000000, -0.000000000000000000 ) ) ;
#78163=ORIENTED_EDGE ( 'NONE', *, *, #70668, .T. ) ;
#78164=DIRECTION ( 'NONE',  ( -4.274815082592931898E-19, -0.9999939076577903929, -0.003490651415223739937 ) ) ;
#78165=VECTOR ( 'NONE', #99016, 1000.000000000000000 ) ;
#78166=AXIS2_PLACEMENT_3D ( 'NONE', #93043, #3995, #112681 ) ;
#78167=VERTEX_POINT ( 'NONE', #28155 ) ;
#78168=CARTESIAN_POINT ( 'NONE',  ( -11.89999999999999680, 2.500000000000000000, -4.083716857408424161 ) ) ;
#78169=VERTEX_POINT ( 'NONE', #68068 ) ;
#78170=DIRECTION ( 'NONE',  ( -0.000000000000000000, -1.000000000000000000, -0.000000000000000000 ) ) ;
#78171=CARTESIAN_POINT ( 'NONE',  ( -3.750000000000025757, 12.50000000000000000, 1.537336459617582918 ) ) ;
#78172=ORIENTED_EDGE ( 'NONE', *, *, #21384, .F. ) ;
#78173=DIRECTION ( 'NONE',  ( 0.000000000000000000, 0.000000000000000000, 1.000000000000000000 ) ) ;
#78174=DIRECTION ( 'NONE',  ( 0.000000000000000000, -0.000000000000000000, 1.000000000000000000 ) ) ;
#78175=AXIS2_PLACEMENT_3D ( 'NONE', #86915, #116373, #14924 ) ;
#78176=ORIENTED_EDGE ( 'NONE', *, *, #105794, .T. ) ;
#78177=CIRCLE ( 'NONE', #13303, 0.09999999999999982514 ) ;
#78178=VECTOR ( 'NONE', #12741, 1000.000000000000000 ) ;
#78179=AXIS2_PLACEMENT_3D ( 'NONE', #45531, #35703, #57275 ) ;
#78180=DIRECTION ( 'NONE',  ( 0.000000000000000000, 0.000000000000000000, 1.000000000000000000 ) ) ;
#78181=ORIENTED_EDGE ( 'NONE', *, *, #27350, .F. ) ;
#78182=VERTEX_POINT ( 'NONE', #129603 ) ;
#78183=CARTESIAN_POINT ( 'NONE',  ( -3.100000000000028511, 12.50000000000000000, 0.3464101615137736845 ) ) ;
#78186=AXIS2_PLACEMENT_3D ( 'NONE', #5646, #76984, #65869 ) ;
#78187=DIRECTION ( 'NONE',  ( -0.000000000000000000, 1.000000000000000000, -0.000000000000000000 ) ) ;
#78188=EDGE_CURVE ( 'NONE', #36304, #8747, #2658, .T. ) ;
#78189=PLANE ( 'NONE',  #60454 ) ;
#78190=CONICAL_SURFACE ( 'NONE', #53052, 0.09999999999999982514, 0.003490658503988666988 ) ;
#78191=VECTOR ( 'NONE', #108677, 1000.000000000000000 ) ;
#78192=VECTOR ( 'NONE', #89813, 1000.000000000000000 ) ;
#78193=DIRECTION ( 'NONE',  ( 0.000000000000000000, -0.000000000000000000, 1.000000000000000000 ) ) ;
#78194=AXIS2_PLACEMENT_3D ( 'NONE', #38174, #69554, #17203 ) ;
#78195=VERTEX_POINT ( 'NONE', #49745 ) ;
#78196=CIRCLE ( 'NONE', #38591, 0.06509327318403745899 ) ;
#78197=DIRECTION ( 'NONE',  ( 0.000000000000000000, 0.000000000000000000, 1.000000000000000000 ) ) ;
#78198=CARTESIAN_POINT ( 'NONE',  ( 1.649999999999951505, 2.500000000000000000, -2.757883832488654097 ) ) ;
#78199=ORIENTED_EDGE ( 'NONE', *, *, #42034, .F. ) ;
#78200=ADVANCED_FACE ( 'NONE', ( #90943 ), #71631, .T. ) ;
#78201=DIRECTION ( 'NONE',  ( 0.000000000000000000, 1.000000000000000000, 0.000000000000000000 ) ) ;
#78203=DIRECTION ( 'NONE',  ( 0.000000000000000000, -0.9999939076577903929, 0.003490651415223739937 ) ) ;
#78204=EDGE_CURVE ( 'NONE', #60586, #129244, #84135, .T. ) ;
#78205=CARTESIAN_POINT ( 'NONE',  ( 10.79999999999991367, 2.500000000000000000, 0.09999999999999761857 ) ) ;
#78206=CARTESIAN_POINT ( 'NONE',  ( 0.8499999999999553468, 12.50000000000000000, -2.165063509461101710 ) ) ;
#78207=ORIENTED_EDGE ( 'NONE', *, *, #81972, .F. ) ;
#78208=DIRECTION ( 'NONE',  ( 0.000000000000000000, 0.000000000000000000, -1.000000000000000000 ) ) ;
#78210=AXIS2_PLACEMENT_3D ( 'NONE', #42437, #71900, #1845 ) ;
#78211=CONICAL_SURFACE ( 'NONE', #21683, 0.1000000000000002554, 0.003490658503988666988 ) ;
#78212=VECTOR ( 'NONE', #109157, 1000.000000000000000 ) ;
#78213=EDGE_CURVE ( 'NONE', #123206, #91215, #33984, .T. ) ;
#78214=ORIENTED_EDGE ( 'NONE', *, *, #13191, .T. ) ;
#78215=DIRECTION ( 'NONE',  ( 0.000000000000000000, 1.000000000000000000, 0.000000000000000000 ) ) ;
#78216=CIRCLE ( 'NONE', #71962, 0.1000000000000000472 ) ;
#78217=CIRCLE ( 'NONE', #51037, 0.06509327318403741736 ) ;
#78218=ORIENTED_EDGE ( 'NONE', *, *, #11416, .T. ) ;
#78219=VECTOR ( 'NONE', #27787, 1000.000000000000000 ) ;
#78220=EDGE_LOOP ( 'NONE', ( #79333, #63326 ) ) ;
#78221=DIRECTION ( 'NONE',  ( 0.000000000000000000, 0.000000000000000000, 1.000000000000000000 ) ) ;
#78222=VECTOR ( 'NONE', #29840, 1000.000000000000000 ) ;
#78223=ORIENTED_EDGE ( 'NONE', *, *, #119633, .F. ) ;
#78224=DIRECTION ( 'NONE',  ( 0.000000000000000000, 0.000000000000000000, 1.000000000000000000 ) ) ;
#78225=CARTESIAN_POINT ( 'NONE',  ( 12.49999999999993960, 2.500000000000000000, 4.230127018922196669 ) ) ;
#78226=DIRECTION ( 'NONE',  ( 0.000000000000000000, 0.000000000000000000, -1.000000000000000000 ) ) ;
#78227=AXIS2_PLACEMENT_3D ( 'NONE', #110550, #71936, #61477 ) ;
#78228=EDGE_LOOP ( 'NONE', ( #52886, #16362 ) ) ;
#78229=AXIS2_PLACEMENT_3D ( 'NONE', #96173, #3931, #6473 ) ;
#78230=AXIS2_PLACEMENT_3D ( 'NONE', #12545, #93699, #100927 ) ;
#78231=DIRECTION ( 'NONE',  ( -0.000000000000000000, -1.000000000000000000, -0.000000000000000000 ) ) ;
#78232=DIRECTION ( 'NONE',  ( 0.000000000000000000, 0.000000000000000000, -1.000000000000000000 ) ) ;
#78233=ORIENTED_EDGE ( 'NONE', *, *, #92673, .F. ) ;
#78234=CONICAL_SURFACE ( 'NONE', #51050, 0.1000000000000000472, 0.003490658503988666988 ) ;
#78235=LINE ( 'NONE', #19950, #71615 ) ;
#78236=DIRECTION ( 'NONE',  ( 0.000000000000000000, -0.9999939076577903929, 0.003490651415223739937 ) ) ;
#78237=ORIENTED_EDGE ( 'NONE', *, *, #2090, .T. ) ;
#78238=EDGE_CURVE ( 'NONE', #66570, #54324, #48658, .T. ) ;
#78239=ORIENTED_EDGE ( 'NONE', *, *, #3121, .F. ) ;
#78240=ORIENTED_EDGE ( 'NONE', *, *, #55455, .T. ) ;
#78241=CARTESIAN_POINT ( 'NONE',  ( 12.69999999999990337, 2.500000000000000000, -4.676537180435978769 ) ) ;
#78242=CARTESIAN_POINT ( 'NONE',  ( 8.349999999999919709, 2.500000000000000000, -1.372243186433550033 ) ) ;
#78243=FACE_OUTER_BOUND ( 'NONE', #103891, .T. ) ;
#78244=EDGE_CURVE ( 'NONE', #68434, #123664, #88333, .T. ) ;
#78245=FACE_BOUND ( 'NONE', #57483, .T. ) ;
#78247=EDGE_CURVE ( 'NONE', #112782, #29210, #15174, .T. ) ;
#78248=ADVANCED_FACE ( 'NONE', ( #3843 ), #72599, .T. ) ;
#78249=DIRECTION ( 'NONE',  ( 0.000000000000000000, 0.000000000000000000, 1.000000000000000000 ) ) ;
#78250=CARTESIAN_POINT ( 'NONE',  ( -8.100000000000010303, 2.500000000000000000, 4.576537180435972019 ) ) ;
#78251=AXIS2_PLACEMENT_3D ( 'NONE', #56315, #15743, #67402 ) ;
#78252=ORIENTED_EDGE ( 'NONE', *, *, #87201, .T. ) ;
#78253=LINE ( 'NONE', #118800, #96708 ) ;
#78254=DIRECTION ( 'NONE',  ( -4.274815082592931898E-19, -0.9999939076577903929, -0.003490651415223739937 ) ) ;
#78255=ADVANCED_FACE ( 'NONE', ( #121678 ), #32695, .T. ) ;
#78256=DIRECTION ( 'NONE',  ( 0.000000000000000000, 0.000000000000000000, -1.000000000000000000 ) ) ;
#78257=LINE ( 'NONE', #99177, #73879 ) ;
#78258=EDGE_CURVE ( 'NONE', #98580, #84166, #51675, .T. ) ;
#78259=DIRECTION ( 'NONE',  ( 0.000000000000000000, 0.000000000000000000, 1.000000000000000000 ) ) ;
#78260=EDGE_CURVE ( 'NONE', #107580, #30611, #42400, .T. ) ;
#78261=FACE_OUTER_BOUND ( 'NONE', #8613, .T. ) ;
#78262=CARTESIAN_POINT ( 'NONE',  ( -10.20000000000000462, 12.50000000000000000, -4.676537180435973440 ) ) ;
#78263=CIRCLE ( 'NONE', #55270, 0.09999999999999982514 ) ;
#78264=CONICAL_SURFACE ( 'NONE', #128447, 0.1000000000000002554, 0.003490658503988666988 ) ;
#78265=EDGE_CURVE ( 'NONE', #4566, #40462, #91585, .T. ) ;
#78266=ORIENTED_EDGE ( 'NONE', *, *, #91256, .F. ) ;
#78267=EDGE_LOOP ( 'NONE', ( #108973, #28783, #105947, #57432 ) ) ;
#78268=ORIENTED_EDGE ( 'NONE', *, *, #98807, .F. ) ;
#78269=ORIENTED_EDGE ( 'NONE', *, *, #101197, .T. ) ;
#78270=ORIENTED_EDGE ( 'NONE', *, *, #72897, .T. ) ;
#78271=CARTESIAN_POINT ( 'NONE',  ( -12.09999999999999609, 12.50000000000000000, -3.637306695894647390 ) ) ;
#78272=LINE ( 'NONE', #37692, #42607 ) ;
#78273=ORIENTED_EDGE ( 'NONE', *, *, #47915, .F. ) ;
#78274=EDGE_CURVE ( 'NONE', #41297, #27877, #17222, .T. ) ;
#78275=FACE_BOUND ( 'NONE', #119509, .T. ) ;
#78276=EDGE_CURVE ( 'NONE', #26093, #24306, #1905, .T. ) ;
#78277=CARTESIAN_POINT ( 'NONE',  ( -2.500000000000030642, 12.50000000000000000, -0.7579135962115916003 ) ) ;
#78278=CIRCLE ( 'NONE', #59510, 0.06509327318403741736 ) ;
#78280=DIRECTION ( 'NONE',  ( 0.000000000000000000, 1.000000000000000000, 0.000000000000000000 ) ) ;
#78281=DIRECTION ( 'NONE',  ( -0.000000000000000000, -1.000000000000000000, -0.000000000000000000 ) ) ;
#78282=CARTESIAN_POINT ( 'NONE',  ( -3.350000000000031619, 12.50000000000000000, -5.802370205355749988 ) ) ;
#78283=VERTEX_POINT ( 'NONE', #2539 ) ;
#78284=DIRECTION ( 'NONE',  ( 0.000000000000000000, -0.9999939076577903929, 0.003490651415223739937 ) ) ;
#78285=VERTEX_POINT ( 'NONE', #102680 ) ;
#78286=VECTOR ( 'NONE', #13814, 1000.000000000000000 ) ;
#78287=CONICAL_SURFACE ( 'NONE', #44834, 0.1000000000000000472, 0.003490658503988666988 ) ;
#78288=EDGE_LOOP ( 'NONE', ( #106025, #26295 ) ) ;
#78289=VERTEX_POINT ( 'NONE', #33959 ) ;
#78290=DIRECTION ( 'NONE',  ( 0.000000000000000000, 0.000000000000000000, -1.000000000000000000 ) ) ;
#78291=DIRECTION ( 'NONE',  ( 0.000000000000000000, 0.000000000000000000, 1.000000000000000000 ) ) ;
#78292=CARTESIAN_POINT ( 'NONE',  ( 12.49999999999993960, 2.500000000000000000, 4.430127018922196847 ) ) ;
#78293=VECTOR ( 'NONE', #56355, 1000.000000000000000 ) ;
#78294=VERTEX_POINT ( 'NONE', #42502 ) ;
#78295=FACE_OUTER_BOUND ( 'NONE', #90319, .T. ) ;
#78296=AXIS2_PLACEMENT_3D ( 'NONE', #82095, #122030, #89972 ) ;
#78297=CARTESIAN_POINT ( 'NONE',  ( 4.349999999999936584, 2.500000000000000000, 6.048780366869520364 ) ) ;
#78298=DIRECTION ( 'NONE',  ( 0.000000000000000000, 1.000000000000000000, 0.000000000000000000 ) ) ;
#78300=DIRECTION ( 'NONE',  ( 0.000000000000000000, 0.000000000000000000, -1.000000000000000000 ) ) ;
#78301=CARTESIAN_POINT ( 'NONE',  ( 7.899999999999924860, 12.50000000000000000, -5.088040615133791356 ) ) ;
#78302=CARTESIAN_POINT ( 'NONE',  ( -5.000000000000024869, 12.50000000000000000, -5.022947341949754119 ) ) ;
#78303=ORIENTED_EDGE ( 'NONE', *, *, #123019, .T. ) ;
#78304=DIRECTION ( 'NONE',  ( 0.000000000000000000, 0.000000000000000000, 1.000000000000000000 ) ) ;
#78305=EDGE_LOOP ( 'NONE', ( #56971, #82477 ) ) ;
#78306=EDGE_CURVE ( 'NONE', #68006, #68510, #92561, .T. ) ;
#78307=CIRCLE ( 'NONE', #103625, 0.09999999999999982514 ) ;
#78309=DIRECTION ( 'NONE',  ( -0.000000000000000000, 1.000000000000000000, -0.000000000000000000 ) ) ;
#78310=AXIS2_PLACEMENT_3D ( 'NONE', #9590, #118897, #29875 ) ;
#78311=ADVANCED_FACE ( 'NONE', ( #12998 ), #27709, .T. ) ;
#78312=DIRECTION ( 'NONE',  ( 0.000000000000000000, 1.000000000000000000, 0.000000000000000000 ) ) ;
#78313=CONICAL_SURFACE ( 'NONE', #11484, 0.09999999999999982514, 0.003490658503988666988 ) ;
#78314=CARTESIAN_POINT ( 'NONE',  ( 1.649999999999948841, 2.500000000000000000, 6.395190528383296602 ) ) ;
#78315=VERTEX_POINT ( 'NONE', #23484 ) ;
#78316=ORIENTED_EDGE ( 'NONE', *, *, #45128, .T. ) ;
#78317=CARTESIAN_POINT ( 'NONE',  ( 6.449999999999931788, 2.500000000000000000, -6.248780366869526759 ) ) ;
#78318=AXIS2_PLACEMENT_3D ( 'NONE', #18372, #40628, #128361 ) ;
#78319=CIRCLE ( 'NONE', #21882, 0.06509327318403741736 ) ;
#78320=PLANE ( 'NONE',  #28646 ) ;
#78321=DIRECTION ( 'NONE',  ( 1.000000000000000000, 0.000000000000000000, 0.000000000000000000 ) ) ;
#78322=ORIENTED_EDGE ( 'NONE', *, *, #237, .F. ) ;
#78323=EDGE_LOOP ( 'NONE', ( #102956, #9844 ) ) ;
#78324=AXIS2_PLACEMENT_3D ( 'NONE', #128269, #98780, #66743 ) ;
#78327=DIRECTION ( 'NONE',  ( 0.000000000000000000, 0.000000000000000000, -1.000000000000000000 ) ) ;
#78328=AXIS2_PLACEMENT_3D ( 'NONE', #77822, #128897, #99427 ) ;
#78329=CIRCLE ( 'NONE', #82530, 0.06509327318403745899 ) ;
#78330=DIRECTION ( 'NONE',  ( -4.274815082592931898E-19, -0.9999939076577903929, -0.003490651415223739937 ) ) ;
#78331=EDGE_LOOP ( 'NONE', ( #7545, #48635, #109251, #128398 ) ) ;
#78332=DIRECTION ( 'NONE',  ( -4.274815082592931898E-19, -0.9999939076577903929, -0.003490651415223739937 ) ) ;
#78333=DIRECTION ( 'NONE',  ( 0.000000000000000000, 0.000000000000000000, -1.000000000000000000 ) ) ;
#78335=DIRECTION ( 'NONE',  ( -0.000000000000000000, -1.000000000000000000, -0.000000000000000000 ) ) ;
#78336=VERTEX_POINT ( 'NONE', #64058 ) ;
#78337=LINE ( 'NONE', #17442, #121991 ) ;
#78338=ORIENTED_EDGE ( 'NONE', *, *, #31447, .T. ) ;
#78339=ORIENTED_EDGE ( 'NONE', *, *, #124329, .T. ) ;
#78340=DIRECTION ( 'NONE',  ( 0.000000000000000000, 1.000000000000000000, 0.000000000000000000 ) ) ;
#78341=DIRECTION ( 'NONE',  ( 0.000000000000000000, 0.000000000000000000, -1.000000000000000000 ) ) ;
#78342=DIRECTION ( 'NONE',  ( 0.000000000000000000, 1.000000000000000000, 0.000000000000000000 ) ) ;
#78343=DIRECTION ( 'NONE',  ( 0.000000000000000000, 1.000000000000000000, 0.000000000000000000 ) ) ;
#78344=AXIS2_PLACEMENT_3D ( 'NONE', #20064, #96343, #105544 ) ;
#78345=DIRECTION ( 'NONE',  ( 0.000000000000000000, 1.000000000000000000, 0.000000000000000000 ) ) ;
#78346=DIRECTION ( 'NONE',  ( -0.000000000000000000, -1.000000000000000000, -0.000000000000000000 ) ) ;
#78347=EDGE_CURVE ( 'NONE', #83000, #74312, #14296, .T. ) ;
#78348=DIRECTION ( 'NONE',  ( 0.000000000000000000, -0.000000000000000000, 1.000000000000000000 ) ) ;
#78349=CARTESIAN_POINT ( 'NONE',  ( 7.899999999999924860, 12.50000000000000000, 3.637306695894644726 ) ) ;
#78350=LINE ( 'NONE', #80276, #33828 ) ;
#78351=DIRECTION ( 'NONE',  ( -0.000000000000000000, -1.000000000000000000, -0.000000000000000000 ) ) ;
#78352=CIRCLE ( 'NONE', #118041, 0.1000000000000000472 ) ;
#78353=ADVANCED_FACE ( 'NONE', ( #44415 ), #514, .T. ) ;
#78354=CONICAL_SURFACE ( 'NONE', #94977, 0.09999999999999999167, 0.003490658503988666988 ) ;
#78355=ORIENTED_EDGE ( 'NONE', *, *, #40578, .F. ) ;
#78356=DIRECTION ( 'NONE',  ( 0.000000000000000000, 0.000000000000000000, 1.000000000000000000 ) ) ;
#78357=ADVANCED_FACE ( 'NONE', ( #54242 ), #123606, .T. ) ;
#78358=CARTESIAN_POINT ( 'NONE',  ( -5.000000000000022204, 2.500000000000000000, 3.637306695894644726 ) ) ;
#78359=LINE ( 'NONE', #7653, #72607 ) ;
#78360=EDGE_CURVE ( 'NONE', #79693, #54054, #4708, .T. ) ;
#78361=PLANE ( 'NONE',  #60960 ) ;
#78362=CARTESIAN_POINT ( 'NONE',  ( -2.900000000000030553, 12.50000000000000000, 4.957854068765711553 ) ) ;
#78363=ORIENTED_EDGE ( 'NONE', *, *, #64795, .F. ) ;
#78364=DIRECTION ( 'NONE',  ( -0.000000000000000000, -1.000000000000000000, -0.000000000000000000 ) ) ;
#78365=AXIS2_PLACEMENT_3D ( 'NONE', #118614, #88500, #38801 ) ;
#78366=EDGE_CURVE ( 'NONE', #29851, #2948, #115625, .T. ) ;
#78367=CIRCLE ( 'NONE', #69949, 0.06509327318403745899 ) ;
#78368=DIRECTION ( 'NONE',  ( 0.000000000000000000, 1.000000000000000000, 0.000000000000000000 ) ) ;
#78369=DIRECTION ( 'NONE',  ( -4.274815082592931898E-19, -0.9999939076577903929, -0.003490651415223739937 ) ) ;
#78370=EDGE_LOOP ( 'NONE', ( #55753, #128377 ) ) ;
#78371=EDGE_CURVE ( 'NONE', #87315, #60348, #84233, .T. ) ;
#78372=ORIENTED_EDGE ( 'NONE', *, *, #49018, .F. ) ;
#78373=DIRECTION ( 'NONE',  ( 0.000000000000000000, 1.000000000000000000, 0.000000000000000000 ) ) ;
#78374=VECTOR ( 'NONE', #87070, 1000.000000000000000 ) ;
#78375=CONICAL_SURFACE ( 'NONE', #116010, 0.09999999999999982514, 0.003490658503988666988 ) ;
#78376=ORIENTED_EDGE ( 'NONE', *, *, #58726, .F. ) ;
#78377=ORIENTED_EDGE ( 'NONE', *, *, #28699, .F. ) ;
#78378=ORIENTED_EDGE ( 'NONE', *, *, #123420, .F. ) ;
#78379=CARTESIAN_POINT ( 'NONE',  ( 8.349999999999923261, 2.500000000000000000, 1.372243186433545370 ) ) ;
#78380=CONICAL_SURFACE ( 'NONE', #111525, 0.09999999999999999167, 0.003490658503988666988 ) ;
#78381=DIRECTION ( 'NONE',  ( 0.000000000000000000, 0.000000000000000000, 1.000000000000000000 ) ) ;
#78382=CARTESIAN_POINT ( 'NONE',  ( -9.200000000000006395, 12.50000000000000000, 4.330127018922196314 ) ) ;
#78383=CIRCLE ( 'NONE', #88824, 0.06509327318403745899 ) ;
#78384=DIRECTION ( 'NONE',  ( 0.000000000000000000, 1.000000000000000000, 0.000000000000000000 ) ) ;
#78385=VERTEX_POINT ( 'NONE', #82430 ) ;
#78386=DIRECTION ( 'NONE',  ( 0.000000000000000000, 1.000000000000000000, 0.000000000000000000 ) ) ;
#78388=DIRECTION ( 'NONE',  ( -0.000000000000000000, 1.000000000000000000, -0.000000000000000000 ) ) ;
#78389=CARTESIAN_POINT ( 'NONE',  ( 17.29982614914525740, -2.489966891809380911, -2.989943721786608943 ) ) ;
#78390=FACE_OUTER_BOUND ( 'NONE', #119254, .T. ) ;
#78391=CARTESIAN_POINT ( 'NONE',  ( -11.05000000000000071, 2.500000000000000000, 6.841600689897072485 ) ) ;
#78392=CARTESIAN_POINT ( 'NONE',  ( 9.549999999999915445, 2.500000000000000000, -2.165063509461101710 ) ) ;
#78393=ORIENTED_EDGE ( 'NONE', *, *, #74734, .T. ) ;
#78394=EDGE_CURVE ( 'NONE', #2954, #72494, #33333, .T. ) ;
#78395=CIRCLE ( 'NONE', #38699, 0.06509327318403745899 ) ;
#78396=VERTEX_POINT ( 'NONE', #83705 ) ;
#78397=ORIENTED_EDGE ( 'NONE', *, *, #116187, .T. ) ;
#78398=AXIS2_PLACEMENT_3D ( 'NONE', #86190, #126135, #76402 ) ;
#78399=ORIENTED_EDGE ( 'NONE', *, *, #58048, .F. ) ;
#78400=EDGE_LOOP ( 'NONE', ( #29955, #104588 ) ) ;
#78401=LINE ( 'NONE', #127492, #92187 ) ;
#78402=CARTESIAN_POINT ( 'NONE',  ( -10.65000000000000213, 12.50000000000000000, 6.213873640053558134 ) ) ;
#78403=CIRCLE ( 'NONE', #19906, 0.1000000000000000472 ) ;
#78404=DIRECTION ( 'NONE',  ( 0.000000000000000000, 0.000000000000000000, 1.000000000000000000 ) ) ;
#78405=EDGE_CURVE ( 'NONE', #13448, #70324, #27800, .T. ) ;
#78406=FACE_BOUND ( 'NONE', #25572, .T. ) ;
#78407=DIRECTION ( 'NONE',  ( 0.000000000000000000, 0.000000000000000000, 1.000000000000000000 ) ) ;
#78408=DIRECTION ( 'NONE',  ( 0.000000000000000000, -0.000000000000000000, 1.000000000000000000 ) ) ;
#78409=EDGE_CURVE ( 'NONE', #55871, #121543, #71422, .T. ) ;
#78410=CARTESIAN_POINT ( 'NONE',  ( -4.800000000000022915, 12.50000000000000000, 3.918623584224382839 ) ) ;
#78411=DIRECTION ( 'NONE',  ( 0.000000000000000000, 0.000000000000000000, 1.000000000000000000 ) ) ;
#78412=AXIS2_PLACEMENT_3D ( 'NONE', #116283, #116925, #5043 ) ;
#78413=CONICAL_SURFACE ( 'NONE', #90911, 0.1000000000000000472, 0.003490658503988666988 ) ;
#78414=AXIS2_PLACEMENT_3D ( 'NONE', #113568, #44174, #16631 ) ;
#78415=ADVANCED_FACE ( 'NONE', ( #126199 ), #96723, .T. ) ;
#78417=AXIS2_PLACEMENT_3D ( 'NONE', #75128, #52917, #92850 ) ;
#78418=ADVANCED_FACE ( 'NONE', ( #95455 ), #111129, .T. ) ;
#78419=DIRECTION ( 'NONE',  ( 0.000000000000000000, 0.000000000000000000, 1.000000000000000000 ) ) ;
#78420=EDGE_CURVE ( 'NONE', #120360, #41032, #59227, .T. ) ;
#78421=DIRECTION ( 'NONE',  ( 0.000000000000000000, -0.9999939076577903929, 0.003490651415223739937 ) ) ;
#78422=ADVANCED_FACE ( 'NONE', ( #106550 ), #25447, .T. ) ;
#78423=VECTOR ( 'NONE', #37757, 1000.000000000000000 ) ;
#78424=AXIS2_PLACEMENT_3D ( 'NONE', #72954, #34335, #113511 ) ;
#78425=DIRECTION ( 'NONE',  ( 0.000000000000000000, -0.000000000000000000, 1.000000000000000000 ) ) ;
#78426=ADVANCED_FACE ( 'NONE', ( #36551 ), #14971, .T. ) ;
#78427=EDGE_LOOP ( 'NONE', ( #68960, #46608 ) ) ;
#78428=VERTEX_POINT ( 'NONE', #107193 ) ;
#78429=EDGE_LOOP ( 'NONE', ( #60589, #8515 ) ) ;
#78430=EDGE_LOOP ( 'NONE', ( #61966, #93846 ) ) ;
#78431=AXIS2_PLACEMENT_3D ( 'NONE', #74156, #44696, #25048 ) ;
#78432=CARTESIAN_POINT ( 'NONE',  ( -8.150000000000012790, 2.500000000000000000, -1.718653347947326049 ) ) ;
#78433=FACE_OUTER_BOUND ( 'NONE', #122479, .T. ) ;
#78434=FACE_BOUND ( 'NONE', #2093, .T. ) ;
#78435=EDGE_CURVE ( 'NONE', #77344, #17860, #92659, .T. ) ;
#78436=CARTESIAN_POINT ( 'NONE',  ( 2.500000000000002220, -2.500000000000000000, 9.000000000000001776 ) ) ;
#78437=ORIENTED_EDGE ( 'NONE', *, *, #116175, .F. ) ;
#78438=DIRECTION ( 'NONE',  ( 0.000000000000000000, 0.000000000000000000, -1.000000000000000000 ) ) ;
#78439=DIRECTION ( 'NONE',  ( 0.000000000000000000, 0.000000000000000000, -1.000000000000000000 ) ) ;
#78440=DIRECTION ( 'NONE',  ( 0.000000000000000000, 0.000000000000000000, 1.000000000000000000 ) ) ;
#78441=DIRECTION ( 'NONE',  ( 0.000000000000000000, 0.000000000000000000, 1.000000000000000000 ) ) ;
#78442=CONICAL_SURFACE ( 'NONE', #70019, 0.09999999999999982514, 0.003490658503988666988 ) ;
#78443=VERTEX_POINT ( 'NONE', #94807 ) ;
#78444=CARTESIAN_POINT ( 'NONE',  ( 12.49999999999990230, 12.50000000000000000, -0.6928203230275541413 ) ) ;
#78445=ORIENTED_EDGE ( 'NONE', *, *, #3345, .F. ) ;
#78446=ORIENTED_EDGE ( 'NONE', *, *, #43528, .F. ) ;
#78447=DIRECTION ( 'NONE',  ( 0.000000000000000000, 0.000000000000000000, 1.000000000000000000 ) ) ;
#78448=DIRECTION ( 'NONE',  ( 0.000000000000000000, 0.000000000000000000, 1.000000000000000000 ) ) ;
#78449=EDGE_LOOP ( 'NONE', ( #93747, #3094, #32991, #125320 ) ) ;
#78450=VECTOR ( 'NONE', #121404, 1000.000000000000000 ) ;
#78451=VECTOR ( 'NONE', #106555, 1000.000000000000000 ) ;
#78452=CARTESIAN_POINT ( 'NONE',  ( 6.449999999999931788, 12.50000000000000000, 6.148780366869520009 ) ) ;
#78453=CARTESIAN_POINT ( 'NONE',  ( -14.39999999999998614, 2.500000000000000000, 0.2464101615137758439 ) ) ;
#78454=ORIENTED_EDGE ( 'NONE', *, *, #29397, .T. ) ;
#78455=CARTESIAN_POINT ( 'NONE',  ( 13.14999999999990088, 12.50000000000000000, 2.511473670974873507 ) ) ;
#78456=ORIENTED_EDGE ( 'NONE', *, *, #33682, .F. ) ;
#78457=DIRECTION ( 'NONE',  ( 0.000000000000000000, 0.000000000000000000, 1.000000000000000000 ) ) ;
#78458=EDGE_LOOP ( 'NONE', ( #70325, #128130, #100191, #120944 ) ) ;
#78459=DIRECTION ( 'NONE',  ( 0.000000000000000000, 0.000000000000000000, 1.000000000000000000 ) ) ;
#78460=FACE_BOUND ( 'NONE', #55061, .T. ) ;
#78461=AXIS2_PLACEMENT_3D ( 'NONE', #25549, #94967, #96878 ) ;
#78462=EDGE_LOOP ( 'NONE', ( #125909, #34764 ) ) ;
#78463=EDGE_CURVE ( 'NONE', #48770, #71603, #40353, .T. ) ;
#78464=AXIS2_PLACEMENT_3D ( 'NONE', #112556, #81159, #121077 ) ;
#78466=VERTEX_POINT ( 'NONE', #75170 ) ;
#78467=CARTESIAN_POINT ( 'NONE',  ( 0.6499999999999561684, 2.500000000000000000, 1.818653347947321475 ) ) ;
#78468=CARTESIAN_POINT ( 'NONE',  ( -2.700000000000030376, 2.500000000000000000, 4.083716857408421497 ) ) ;
#78469=CARTESIAN_POINT ( 'NONE',  ( 10.19999999999991580, 2.500000000000000000, -0.3464101615137783474 ) ) ;
#78470=DIRECTION ( 'NONE',  ( 0.000000000000000000, 1.000000000000000000, 0.000000000000000000 ) ) ;
#78471=DIRECTION ( 'NONE',  ( -0.000000000000000000, -1.000000000000000000, -0.000000000000000000 ) ) ;
#78472=ORIENTED_EDGE ( 'NONE', *, *, #47074, .F. ) ;
#78473=EDGE_LOOP ( 'NONE', ( #72109, #46407, #62712, #91992 ) ) ;
#78474=ADVANCED_FACE ( 'NONE', ( #115067 ), #123943, .T. ) ;
#78475=ORIENTED_EDGE ( 'NONE', *, *, #101435, .F. ) ;
#78476=DIRECTION ( 'NONE',  ( -0.000000000000000000, 1.000000000000000000, -0.000000000000000000 ) ) ;
#78477=VECTOR ( 'NONE', #53302, 1000.000000000000000 ) ;
#78478=CIRCLE ( 'NONE', #22033, 0.1000000000000002554 ) ;
#78479=CARTESIAN_POINT ( 'NONE',  ( 8.749999999999921840, 12.50000000000000000, 2.857883832488649301 ) ) ;
#78480=CARTESIAN_POINT ( 'NONE',  ( 12.69999999999990159, 12.50000000000000000, -3.983716857408426293 ) ) ;
#78481=VERTEX_POINT ( 'NONE', #37189 ) ;
#78482=EDGE_LOOP ( 'NONE', ( #72431, #112664, #386, #69579 ) ) ;
#78483=ORIENTED_EDGE ( 'NONE', *, *, #85001, .F. ) ;
#78484=DIRECTION ( 'NONE',  ( 0.000000000000000000, 0.000000000000000000, -1.000000000000000000 ) ) ;
#78485=CARTESIAN_POINT ( 'NONE',  ( 1.449999999999952216, 12.50000000000000000, -2.511473670974877948 ) ) ;
#78486=DIRECTION ( 'NONE',  ( -0.000000000000000000, -1.000000000000000000, -0.000000000000000000 ) ) ;
#78487=CARTESIAN_POINT ( 'NONE',  ( -5.200000000000024158, 12.50000000000000000, -4.676537180435977881 ) ) ;
#78488=VECTOR ( 'NONE', #23372, 1000.000000000000000 ) ;
#78489=DIRECTION ( 'NONE',  ( -0.000000000000000000, 1.000000000000000000, -0.000000000000000000 ) ) ;
#78490=CARTESIAN_POINT ( 'NONE',  ( -11.64999999999999680, 12.50000000000000000, -6.495190528383298911 ) ) ;
#78491=FACE_OUTER_BOUND ( 'NONE', #38910, .T. ) ;
#78492=AXIS2_PLACEMENT_3D ( 'NONE', #117723, #86338, #126285 ) ;
#78493=CARTESIAN_POINT ( 'NONE',  ( 10.19999999999991402, 2.500000000000000000, 0.3464101615137735735 ) ) ;
#78494=ORIENTED_EDGE ( 'NONE', *, *, #12907, .T. ) ;
#78495=VERTEX_POINT ( 'NONE', #65986 ) ;
#78496=CARTESIAN_POINT ( 'NONE',  ( -12.89999999999999147, 2.500000000000000000, -0.09999999999999815981 ) ) ;
#78497=AXIS2_PLACEMENT_3D ( 'NONE', #122291, #32642, #83013 ) ;
#78498=AXIS2_PLACEMENT_3D ( 'NONE', #105712, #94579, #65112 ) ;
#78499=DIRECTION ( 'NONE',  ( 0.000000000000000000, 0.000000000000000000, -1.000000000000000000 ) ) ;
#78500=ORIENTED_EDGE ( 'NONE', *, *, #73991, .T. ) ;
#78501=( BOUNDED_CURVE ( )  B_SPLINE_CURVE ( 2, ( #123862, #104860, #3458 ),
 .UNSPECIFIED., .F., .F. ) 
 B_SPLINE_CURVE_WITH_KNOTS ( ( 3, 3 ),
 ( 0.000000000000000000, 0.01492713794235515402 ),
 .UNSPECIFIED. ) 
 CURVE ( )  GEOMETRIC_REPRESENTATION_ITEM ( )  RATIONAL_B_SPLINE_CURVE ( ( 0.8943752373141968803, 0.7762344340431479583, 1.000000000000000000 ) ) 
 REPRESENTATION_ITEM ( '' )  );
#78502=EDGE_LOOP ( 'NONE', ( #64012, #12238 ) ) ;
#78504=CARTESIAN_POINT ( 'NONE',  ( -8.150000000000012790, 12.50000000000000000, -1.883746621131363597 ) ) ;
#78505=DIRECTION ( 'NONE',  ( 0.000000000000000000, 1.000000000000000000, 0.000000000000000000 ) ) ;
#78506=CONICAL_SURFACE ( 'NONE', #95213, 0.09999999999999982514, 0.003490658503988666988 ) ;
#78507=DIRECTION ( 'NONE',  ( -0.000000000000000000, 1.000000000000000000, -0.000000000000000000 ) ) ;
#78508=AXIS2_PLACEMENT_3D ( 'NONE', #117688, #28053, #67961 ) ;
#78509=AXIS2_PLACEMENT_3D ( 'NONE', #10673, #42102, #2162 ) ;
#78510=CARTESIAN_POINT ( 'NONE',  ( -12.29999999999999361, 2.500000000000000000, 3.983716857408420076 ) ) ;
#78511=DIRECTION ( 'NONE',  ( 0.000000000000000000, 0.000000000000000000, 1.000000000000000000 ) ) ;
#78512=DIRECTION ( 'NONE',  ( -0.000000000000000000, -1.000000000000000000, -0.000000000000000000 ) ) ;
#78513=AXIS2_PLACEMENT_3D ( 'NONE', #25211, #101857, #12168 ) ;
#78514=DIRECTION ( 'NONE',  ( 0.000000000000000000, 0.000000000000000000, 1.000000000000000000 ) ) ;
#78515=AXIS2_PLACEMENT_3D ( 'NONE', #53387, #33735, #84115 ) ;
#78516=AXIS2_PLACEMENT_3D ( 'NONE', #113357, #52500, #43350 ) ;
#78517=EDGE_CURVE ( 'NONE', #68282, #96334, #121902, .T. ) ;
#78518=EDGE_LOOP ( 'NONE', ( #110738, #97042 ) ) ;
#78519=ORIENTED_EDGE ( 'NONE', *, *, #78889, .F. ) ;
#78520=AXIS2_PLACEMENT_3D ( 'NONE', #88973, #38604, #7819 ) ;
#78521=EDGE_CURVE ( 'NONE', #50743, #118622, #31739, .T. ) ;
#78522=ORIENTED_EDGE ( 'NONE', *, *, #73616, .T. ) ;
#78523=ORIENTED_EDGE ( 'NONE', *, *, #64015, .F. ) ;
#78524=EDGE_CURVE ( 'NONE', #59372, #125242, #105168, .T. ) ;
#78525=CARTESIAN_POINT ( 'NONE',  ( -2.100000000000033840, 12.50000000000000000, 4.957854068765711553 ) ) ;
#78526=LINE ( 'NONE', #88969, #3903 ) ;
#78527=VERTEX_POINT ( 'NONE', #56783 ) ;
#78528=DIRECTION ( 'NONE',  ( 0.000000000000000000, 0.000000000000000000, -1.000000000000000000 ) ) ;
#78529=FACE_OUTER_BOUND ( 'NONE', #40009, .T. ) ;
#78530=EDGE_CURVE ( 'NONE', #51256, #82532, #4805, .T. ) ;
#78531=DIRECTION ( 'NONE',  ( 0.000000000000000000, 0.000000000000000000, 1.000000000000000000 ) ) ;
#78532=CARTESIAN_POINT ( 'NONE',  ( -2.500000000000032419, 2.500000000000000000, 0.5928203230275495006 ) ) ;
#78533=EDGE_LOOP ( 'NONE', ( #74164, #68174 ) ) ;
#78534=EDGE_CURVE ( 'NONE', #51476, #12146, #613, .T. ) ;
#78535=DIRECTION ( 'NONE',  ( 0.000000000000000000, 1.000000000000000000, 0.000000000000000000 ) ) ;
#78536=CIRCLE ( 'NONE', #40882, 0.06509327318403745899 ) ;
#78537=FACE_OUTER_BOUND ( 'NONE', #46733, .T. ) ;
#78538=EDGE_LOOP ( 'NONE', ( #95274, #6679 ) ) ;
#78539=ORIENTED_EDGE ( 'NONE', *, *, #12618, .F. ) ;
#78540=VERTEX_POINT ( 'NONE', #17519 ) ;
#78541=PLANE ( 'NONE',  #19535 ) ;
#78542=CIRCLE ( 'NONE', #40891, 0.09999999999999982514 ) ;
#78543=CIRCLE ( 'NONE', #88985, 0.06509327318403745899 ) ;
#78545=CIRCLE ( 'NONE', #30427, 0.06509327318403745899 ) ;
#78546=ORIENTED_EDGE ( 'NONE', *, *, #39599, .T. ) ;
#78547=DIRECTION ( 'NONE',  ( 0.000000000000000000, 1.000000000000000000, 0.000000000000000000 ) ) ;
#78548=CARTESIAN_POINT ( 'NONE',  ( -3.550000000000028244, 2.500000000000000000, -1.718653347947326049 ) ) ;
#78549=CARTESIAN_POINT ( 'NONE',  ( -11.04999999999999893, 2.500000000000000000, 6.148780366869520009 ) ) ;
#78550=DIRECTION ( 'NONE',  ( -0.000000000000000000, -1.000000000000000000, -0.000000000000000000 ) ) ;
#78551=AXIS2_PLACEMENT_3D ( 'NONE', #87703, #117797, #28153 ) ;
#78552=ORIENTED_EDGE ( 'NONE', *, *, #3809, .F. ) ;
#78553=FACE_OUTER_BOUND ( 'NONE', #25142, .T. ) ;
#78554=AXIS2_PLACEMENT_3D ( 'NONE', #29331, #59449, #9677 ) ;
#78555=ORIENTED_EDGE ( 'NONE', *, *, #88429, .F. ) ;
#78556=ORIENTED_EDGE ( 'NONE', *, *, #126777, .F. ) ;
#78557=CARTESIAN_POINT ( 'NONE',  ( -11.69999999999999574, 12.50000000000000000, 4.330127018922196314 ) ) ;
#78558=DIRECTION ( 'NONE',  ( 0.000000000000000000, 0.000000000000000000, 1.000000000000000000 ) ) ;
#78559=FACE_BOUND ( 'NONE', #65201, .T. ) ;
#78560=DIRECTION ( 'NONE',  ( 0.000000000000000000, -0.9999939076577903929, 0.003490651415223739937 ) ) ;
#78561=CARTESIAN_POINT ( 'NONE',  ( -11.64999999999999680, 12.50000000000000000, 1.472243186433545459 ) ) ;
#78562=DIRECTION ( 'NONE',  ( 0.000000000000000000, 0.000000000000000000, 1.000000000000000000 ) ) ;
#78563=AXIS2_PLACEMENT_3D ( 'NONE', #48626, #127820, #70198 ) ;
#78564=AXIS2_PLACEMENT_3D ( 'NONE', #90487, #100959, #20484 ) ;
#78565=ADVANCED_FACE ( 'NONE', ( #114434 ), #21556, .T. ) ;
#78566=ORIENTED_EDGE ( 'NONE', *, *, #66666, .T. ) ;
#78567=EDGE_CURVE ( 'NONE', #51160, #52643, #105271, .T. ) ;
#78568=DIRECTION ( 'NONE',  ( -0.000000000000000000, 1.000000000000000000, -0.000000000000000000 ) ) ;
#78569=CARTESIAN_POINT ( 'NONE',  ( 6.449999999999930012, 2.500000000000000000, 6.941600689897073018 ) ) ;
#78570=DIRECTION ( 'NONE',  ( 0.000000000000000000, 0.000000000000000000, 1.000000000000000000 ) ) ;
#78571=EDGE_CURVE ( 'NONE', #65511, #127177, #36232, .T. ) ;
#78572=DIRECTION ( 'NONE',  ( 0.000000000000000000, 1.000000000000000000, 0.000000000000000000 ) ) ;
#78573=VERTEX_POINT ( 'NONE', #10294 ) ;
#78574=DIRECTION ( 'NONE',  ( -4.274815082592931898E-19, -0.9999939076577903929, -0.003490651415223739937 ) ) ;
#78575=DIRECTION ( 'NONE',  ( 0.000000000000000000, 0.000000000000000000, 1.000000000000000000 ) ) ;
#78576=EDGE_CURVE ( 'NONE', #56898, #45181, #109113, .T. ) ;
#78578=ORIENTED_EDGE ( 'NONE', *, *, #65950, .F. ) ;
#78579=CARTESIAN_POINT ( 'NONE',  ( -4.150000000000024336, 2.500000000000000000, 2.165063509461097713 ) ) ;
#78580=CARTESIAN_POINT ( 'NONE',  ( -3.950000000000026379, 12.50000000000000000, 2.446380397790835826 ) ) ;
#78581=FACE_BOUND ( 'NONE', #76602, .T. ) ;
#78582=CARTESIAN_POINT ( 'NONE',  ( 13.92826131978669224, -2.499999999999998668, -6.790916465128551849 ) ) ;
#78583=EDGE_CURVE ( 'NONE', #54326, #8077, #77987, .T. ) ;
#78584=ADVANCED_FACE ( 'NONE', ( #129454 ), #50807, .T. ) ;
#78585=CONICAL_SURFACE ( 'NONE', #89032, 0.09999999999999982514, 0.003490658503988666988 ) ;
#78586=ORIENTED_EDGE ( 'NONE', *, *, #76192, .T. ) ;
#78587=CARTESIAN_POINT ( 'NONE',  ( -10.20000000000000462, 2.500000000000000000, -4.576537180435972907 ) ) ;
#78588=VECTOR ( 'NONE', #68993, 1000.000000000000000 ) ;
#78589=ORIENTED_EDGE ( 'NONE', *, *, #15496, .F. ) ;
#78590=VERTEX_POINT ( 'NONE', #128139 ) ;
#78591=FACE_OUTER_BOUND ( 'NONE', #100367, .T. ) ;
#78593=EDGE_CURVE ( 'NONE', #108519, #88013, #111420, .T. ) ;
#78594=ORIENTED_EDGE ( 'NONE', *, *, #128348, .F. ) ;
#78595=FACE_OUTER_BOUND ( 'NONE', #43276, .T. ) ;
#78596=CARTESIAN_POINT ( 'NONE',  ( 11.84999999999990372, 2.500000000000000000, 2.611473670974873151 ) ) ;
#78597=VECTOR ( 'NONE', #62440, 1000.000000000000000 ) ;
#78598=FACE_OUTER_BOUND ( 'NONE', #27591, .T. ) ;
#78599=CARTESIAN_POINT ( 'NONE',  ( -10.20000000000000284, 12.50000000000000000, 3.983716857408420964 ) ) ;
#78600=AXIS2_PLACEMENT_3D ( 'NONE', #125736, #126405, #85821 ) ;
#78601=ORIENTED_EDGE ( 'NONE', *, *, #25003, .T. ) ;
#78602=CIRCLE ( 'NONE', #24300, 0.06509327318403745899 ) ;
#78603=DIRECTION ( 'NONE',  ( 0.000000000000000000, 1.000000000000000000, 0.000000000000000000 ) ) ;
#78604=LINE ( 'NONE', #68754, #129152 ) ;
#78605=LINE ( 'NONE', #28198, #109914 ) ;
#78606=CIRCLE ( 'NONE', #38916, 0.1000000000000002554 ) ;
#78607=CARTESIAN_POINT ( 'NONE',  ( 13.09999999999990195, 2.500000000000000000, -4.676537180435978769 ) ) ;
#78608=EDGE_LOOP ( 'NONE', ( #463, #72921, #19313, #13586 ) ) ;
#78609=DIRECTION ( 'NONE',  ( 0.000000000000000000, 0.000000000000000000, 1.000000000000000000 ) ) ;
#78610=ORIENTED_EDGE ( 'NONE', *, *, #5521, .F. ) ;
#78611=DIRECTION ( 'NONE',  ( -0.000000000000000000, 1.000000000000000000, -0.000000000000000000 ) ) ;
#78612=ORIENTED_EDGE ( 'NONE', *, *, #103233, .F. ) ;
#78613=LINE ( 'NONE', #69402, #51129 ) ;
#78614=CARTESIAN_POINT ( 'NONE',  ( 6.649999999999929301, 2.500000000000000000, 6.495190528383297135 ) ) ;
#78617=ORIENTED_EDGE ( 'NONE', *, *, #40895, .T. ) ;
#78618=CARTESIAN_POINT ( 'NONE',  ( 11.24999999999991118, 2.500000000000000000, -2.757883832488654097 ) ) ;
#78619=CARTESIAN_POINT ( 'NONE',  ( -12.29999999999999716, 2.500000000000000000, 0.3464101615137776813 ) ) ;
#78620=DIRECTION ( 'NONE',  ( -4.274815082592931898E-19, -0.9999939076577903929, -0.003490651415223739937 ) ) ;
#78622=CARTESIAN_POINT ( 'NONE',  ( 13.09999999999990195, 2.500000000000000000, 3.883716857408420431 ) ) ;
#78623=VECTOR ( 'NONE', #13040, 1000.000000000000000 ) ;
#78624=DIRECTION ( 'NONE',  ( -0.000000000000000000, 1.000000000000000000, -0.000000000000000000 ) ) ;
#78625=ORIENTED_EDGE ( 'NONE', *, *, #79165, .F. ) ;
#78626=ADVANCED_FACE ( 'NONE', ( #30597 ), #19460, .T. ) ;
#78627=EDGE_LOOP ( 'NONE', ( #71911, #102560 ) ) ;
#78628=DIRECTION ( 'NONE',  ( 0.000000000000000000, 0.000000000000000000, 1.000000000000000000 ) ) ;
#78629=ORIENTED_EDGE ( 'NONE', *, *, #64636, .F. ) ;
#78630=DIRECTION ( 'NONE',  ( -0.000000000000000000, 1.000000000000000000, -0.000000000000000000 ) ) ;
#78631=ORIENTED_EDGE ( 'NONE', *, *, #50450, .F. ) ;
#78632=VERTEX_POINT ( 'NONE', #59419 ) ;
#78633=VECTOR ( 'NONE', #75211, 1000.000000000000000 ) ;
#78634=ORIENTED_EDGE ( 'NONE', *, *, #15659, .F. ) ;
#78635=DIRECTION ( 'NONE',  ( -4.274815082592931898E-19, -0.9999939076577903929, -0.003490651415223739937 ) ) ;
#78636=AXIS2_PLACEMENT_3D ( 'NONE', #29622, #38161, #28348 ) ;
#78637=AXIS2_PLACEMENT_3D ( 'NONE', #123954, #35595, #33657 ) ;
#78638=DIRECTION ( 'NONE',  ( 0.000000000000000000, 0.000000000000000000, 1.000000000000000000 ) ) ;
#78639=DIRECTION ( 'NONE',  ( -0.000000000000000000, -1.000000000000000000, -0.000000000000000000 ) ) ;
#78640=CIRCLE ( 'NONE', #15905, 0.06509327318403745899 ) ;
#78641=DIRECTION ( 'NONE',  ( 0.000000000000000000, 1.000000000000000000, 0.000000000000000000 ) ) ;
#78642=CARTESIAN_POINT ( 'NONE',  ( 1.249999999999950262, 2.500000000000000000, 7.188010851410848723 ) ) ;
#78643=CARTESIAN_POINT ( 'NONE',  ( 3.149999999999944400, 2.500000000000000000, 2.411473670974873862 ) ) ;
#78644=FACE_OUTER_BOUND ( 'NONE', #20886, .T. ) ;
#78645=CARTESIAN_POINT ( 'NONE',  ( 5.199999999999935341, 12.50000000000000000, -4.048810130592463530 ) ) ;
#78646=ORIENTED_EDGE ( 'NONE', *, *, #10800, .T. ) ;
#78647=AXIS2_PLACEMENT_3D ( 'NONE', #110419, #29299, #119587 ) ;
#78648=ORIENTED_EDGE ( 'NONE', *, *, #59633, .F. ) ;
#78649=ORIENTED_EDGE ( 'NONE', *, *, #98802, .F. ) ;
#78650=CIRCLE ( 'NONE', #74428, 0.06509327318403745899 ) ;
#78652=EDGE_LOOP ( 'NONE', ( #39151, #1092, #25931, #79314 ) ) ;
#78653=ORIENTED_EDGE ( 'NONE', *, *, #65818, .T. ) ;
#78654=DIRECTION ( 'NONE',  ( -0.000000000000000000, 1.000000000000000000, -0.000000000000000000 ) ) ;
#78655=DIRECTION ( 'NONE',  ( -0.000000000000000000, 1.000000000000000000, -0.000000000000000000 ) ) ;
#78656=DIRECTION ( 'NONE',  ( -0.000000000000000000, -1.000000000000000000, -0.000000000000000000 ) ) ;
#78657=DIRECTION ( 'NONE',  ( 0.000000000000000000, -0.000000000000000000, 1.000000000000000000 ) ) ;
#78658=CARTESIAN_POINT ( 'NONE',  ( 11.89999999999990798, 12.50000000000000000, -3.983716857408426293 ) ) ;
#78659=ORIENTED_EDGE ( 'NONE', *, *, #541, .T. ) ;
#78660=DIRECTION ( 'NONE',  ( 0.000000000000000000, -0.000000000000000000, 1.000000000000000000 ) ) ;
#78661=EDGE_LOOP ( 'NONE', ( #42064, #88892, #121495, #45648 ) ) ;
#78662=DIRECTION ( 'NONE',  ( -4.274815082592931898E-19, -0.9999939076577903929, -0.003490651415223739937 ) ) ;
#78663=ADVANCED_FACE ( 'NONE', ( #20756 ), #67496, .T. ) ;
#78664=VERTEX_POINT ( 'NONE', #77723 ) ;
#78665=FACE_OUTER_BOUND ( 'NONE', #107510, .T. ) ;
#78666=EDGE_LOOP ( 'NONE', ( #40115, #67024, #2528, #112494 ) ) ;
#78668=ORIENTED_EDGE ( 'NONE', *, *, #74403, .T. ) ;
#78669=EDGE_CURVE ( 'NONE', #19600, #91108, #65454, .T. ) ;
#78670=LINE ( 'NONE', #59014, #92068 ) ;
#78671=CARTESIAN_POINT ( 'NONE',  ( -12.49999999999999289, 2.500000000000000000, -0.6928203230275500335 ) ) ;
#78672=CONICAL_SURFACE ( 'NONE', #105843, 0.1000000000000000472, 0.003490658503988666988 ) ;
#78673=CARTESIAN_POINT ( 'NONE',  ( -1.900000000000034106, 2.500000000000000000, -3.883716857408426648 ) ) ;
#78674=CARTESIAN_POINT ( 'NONE',  ( 6.849999999999929479, 2.500000000000000000, 6.841600689897072485 ) ) ;
#78675=ADVANCED_FACE ( 'NONE', ( #104250 ), #98917, .T. ) ;
#78676=CARTESIAN_POINT ( 'NONE',  ( 0.6499999999999566125, 2.500000000000000000, -6.941600689897077459 ) ) ;
#78677=ADVANCED_FACE ( 'NONE', ( #93152 ), #54691, .T. ) ;
#78678=VERTEX_POINT ( 'NONE', #91211 ) ;
#78679=DIRECTION ( 'NONE',  ( 0.000000000000000000, 1.000000000000000000, 0.000000000000000000 ) ) ;
#78680=CARTESIAN_POINT ( 'NONE',  ( 7.499999999999961808, 2.500000000000000000, 4.430127018922196847 ) ) ;
#78681=ADVANCED_FACE ( 'NONE', ( #3471 ), #71531, .T. ) ;
#78682=DIRECTION ( 'NONE',  ( 0.000000000000000000, 1.000000000000000000, 0.000000000000000000 ) ) ;
#78683=EDGE_CURVE ( 'NONE', #95241, #4391, #67290, .T. ) ;
#78684=EDGE_CURVE ( 'NONE', #113935, #64066, #62408, .T. ) ;
#78685=DIRECTION ( 'NONE',  ( 0.000000000000000000, 0.000000000000000000, 1.000000000000000000 ) ) ;
#78686=CIRCLE ( 'NONE', #24383, 0.1000000000000002554 ) ;
#78687=VECTOR ( 'NONE', #109798, 1000.000000000000000 ) ;
#78688=DIRECTION ( 'NONE',  ( 0.000000000000000000, -0.9999939076577903929, 0.003490651415223739937 ) ) ;
#78689=ORIENTED_EDGE ( 'NONE', *, *, #119160, .F. ) ;
#78690=VERTEX_POINT ( 'NONE', #82694 ) ;
#78691=CARTESIAN_POINT ( 'NONE',  ( 11.84999999999990372, 12.50000000000000000, -6.148780366869526226 ) ) ;
#78692=ADVANCED_FACE ( 'NONE', ( #73484 ), #29683, .T. ) ;
#78693=EDGE_LOOP ( 'NONE', ( #36564, #34636 ) ) ;
#78694=AXIS2_PLACEMENT_3D ( 'NONE', #125190, #25686, #15862 ) ;
#78695=AXIS2_PLACEMENT_3D ( 'NONE', #82587, #11240, #121846 ) ;
#78696=CARTESIAN_POINT ( 'NONE',  ( -7.050000000000016698, 12.50000000000000000, -6.560283801567339701 ) ) ;
#78697=PLANE ( 'NONE',  #64903 ) ;
#78698=CIRCLE ( 'NONE', #105868, 0.06509327318403745899 ) ;
#78699=EDGE_LOOP ( 'NONE', ( #110897, #84263 ) ) ;
#78701=CARTESIAN_POINT ( 'NONE',  ( -8.750000000000010658, 2.500000000000000000, 2.857883832488649301 ) ) ;
#78702=DIRECTION ( 'NONE',  ( -4.274815082592931898E-19, -0.9999939076577903929, -0.003490651415223739937 ) ) ;
#78703=DIRECTION ( 'NONE',  ( 0.000000000000000000, 0.000000000000000000, -1.000000000000000000 ) ) ;
#78704=ORIENTED_EDGE ( 'NONE', *, *, #102482, .F. ) ;
#78705=CARTESIAN_POINT ( 'NONE',  ( 6.249999999999965361, 2.500000000000000000, 2.265063509461097357 ) ) ;
#78706=VERTEX_POINT ( 'NONE', #22493 ) ;
#78707=DIRECTION ( 'NONE',  ( -0.000000000000000000, 1.000000000000000000, -0.000000000000000000 ) ) ;
#78708=AXIS2_PLACEMENT_3D ( 'NONE', #117039, #27374, #67279 ) ;
#78709=DIRECTION ( 'NONE',  ( -4.274815082592931898E-19, -0.9999939076577903929, -0.003490651415223739937 ) ) ;
#78711=VERTEX_POINT ( 'NONE', #32957 ) ;
#78712=AXIS2_PLACEMENT_3D ( 'NONE', #19949, #8809, #99797 ) ;
#78713=CIRCLE ( 'NONE', #53569, 0.06509327318403743123 ) ;
#78714=DIRECTION ( 'NONE',  ( -0.000000000000000000, -1.000000000000000000, -0.000000000000000000 ) ) ;
#78715=CONICAL_SURFACE ( 'NONE', #22291, 0.1000000000000002554, 0.003490658503988666988 ) ;
#78716=ORIENTED_EDGE ( 'NONE', *, *, #70009, .T. ) ;
#78717=EDGE_CURVE ( 'NONE', #38652, #6400, #77774, .T. ) ;
#78718=CARTESIAN_POINT ( 'NONE',  ( 4.149999999999938183, 12.50000000000000000, 7.188010851410848723 ) ) ;
#78719=CARTESIAN_POINT ( 'NONE',  ( 4.999999999999936939, 2.500000000000000000, -0.5928203230275541635 ) ) ;
#78720=VECTOR ( 'NONE', #50893, 1000.000000000000000 ) ;
#78721=LINE ( 'NONE', #118621, #7806 ) ;
#78722=EDGE_CURVE ( 'NONE', #6219, #115023, #23767, .T. ) ;
#78723=AXIS2_PLACEMENT_3D ( 'NONE', #126549, #48630, #116710 ) ;
#78724=VERTEX_POINT ( 'NONE', #44045 ) ;
#78725=CARTESIAN_POINT ( 'NONE',  ( 2.099999999999950351, 2.500000000000000000, -5.022947341949754119 ) ) ;
#78726=AXIS2_PLACEMENT_3D ( 'NONE', #26369, #17141, #117279 ) ;
#78727=EDGE_CURVE ( 'NONE', #115959, #33163, #11998, .T. ) ;
#78728=CARTESIAN_POINT ( 'NONE',  ( -10.20000000000000462, 2.500000000000000000, 0.3464101615137735735 ) ) ;
#78730=DIRECTION ( 'NONE',  ( 0.000000000000000000, 0.000000000000000000, 1.000000000000000000 ) ) ;
#78731=ADVANCED_FACE ( 'NONE', ( #111486 ), #4101, .T. ) ;
#78732=ORIENTED_EDGE ( 'NONE', *, *, #8443, .F. ) ;
#78733=CARTESIAN_POINT ( 'NONE',  ( -11.05000000000000249, 2.500000000000000000, -6.148780366869522673 ) ) ;
#78734=AXIS2_PLACEMENT_3D ( 'NONE', #123932, #4795, #75478 ) ;
#78735=EDGE_CURVE ( 'NONE', #58451, #7794, #66888, .T. ) ;
#78736=EDGE_CURVE ( 'NONE', #27277, #17873, #47272, .T. ) ;
#78737=AXIS2_PLACEMENT_3D ( 'NONE', #97293, #64607, #36465 ) ;
#78738=AXIS2_PLACEMENT_3D ( 'NONE', #78614, #49154, #10484 ) ;
#78739=ADVANCED_FACE ( 'NONE', ( #106191 ), #6649, .T. ) ;
#78740=ORIENTED_EDGE ( 'NONE', *, *, #52986, .T. ) ;
#78741=DIRECTION ( 'NONE',  ( -0.000000000000000000, -1.000000000000000000, -0.000000000000000000 ) ) ;
#78742=CARTESIAN_POINT ( 'NONE',  ( 3.549999999999940314, 12.50000000000000000, 6.841600689897072485 ) ) ;
#78743=ORIENTED_EDGE ( 'NONE', *, *, #77593, .T. ) ;
#78745=DIRECTION ( 'NONE',  ( -0.000000000000000000, -1.000000000000000000, -0.000000000000000000 ) ) ;
#78746=DIRECTION ( 'NONE',  ( 0.000000000000000000, 0.000000000000000000, 1.000000000000000000 ) ) ;
#78747=ORIENTED_EDGE ( 'NONE', *, *, #76084, .T. ) ;
#78748=ADVANCED_FACE ( 'NONE', ( #4733 ), #115415, .T. ) ;
#78749=DIRECTION ( 'NONE',  ( -0.000000000000000000, 1.000000000000000000, -0.000000000000000000 ) ) ;
#78750=CARTESIAN_POINT ( 'NONE',  ( -2.900000000000030109, 2.500000000000000000, -3.737306695894649700 ) ) ;
#78751=DIRECTION ( 'NONE',  ( -0.000000000000000000, -1.000000000000000000, -0.000000000000000000 ) ) ;
#78752=DIRECTION ( 'NONE',  ( -0.000000000000000000, 1.000000000000000000, -0.000000000000000000 ) ) ;
#78753=DIRECTION ( 'NONE',  ( 0.000000000000000000, 1.000000000000000000, 0.000000000000000000 ) ) ;
#78754=LINE ( 'NONE', #9991, #47316 ) ;
#78755=DIRECTION ( 'NONE',  ( 0.000000000000000000, 0.000000000000000000, 1.000000000000000000 ) ) ;
#78756=EDGE_LOOP ( 'NONE', ( #44330, #74518, #42474, #47401 ) ) ;
#78758=VERTEX_POINT ( 'NONE', #35522 ) ;
#78759=ORIENTED_EDGE ( 'NONE', *, *, #40136, .F. ) ;
#78760=FACE_OUTER_BOUND ( 'NONE', #53442, .T. ) ;
#78761=DIRECTION ( 'NONE',  ( 0.000000000000000000, 0.000000000000000000, -1.000000000000000000 ) ) ;
#78762=FACE_OUTER_BOUND ( 'NONE', #56611, .T. ) ;
#78763=EDGE_LOOP ( 'NONE', ( #32442, #59890, #37, #2548 ) ) ;
#78764=FACE_BOUND ( 'NONE', #33950, .T. ) ;
#78766=EDGE_CURVE ( 'NONE', #23542, #87945, #107471, .T. ) ;
#78767=LINE ( 'NONE', #59114, #85628 ) ;
#78768=LINE ( 'NONE', #118662, #97940 ) ;
#78769=CARTESIAN_POINT ( 'NONE',  ( -7.700000000000014388, 12.50000000000000000, -4.611443907251939756 ) ) ;
#78770=CARTESIAN_POINT ( 'NONE',  ( -1.650000000000034328, 2.500000000000000000, -2.065063509461102065 ) ) ;
#78771=AXIS2_PLACEMENT_3D ( 'NONE', #123719, #24255, #54995 ) ;
#78772=CARTESIAN_POINT ( 'NONE',  ( -7.300000000000018474, 2.500000000000000000, -3.983716857408426293 ) ) ;
#78773=CARTESIAN_POINT ( 'NONE',  ( 8.299999999999922551, 12.50000000000000000, 0.06509327318403504425 ) ) ;
#78774=ORIENTED_EDGE ( 'NONE', *, *, #16891, .F. ) ;
#78775=DIRECTION ( 'NONE',  ( 0.000000000000000000, 0.000000000000000000, 1.000000000000000000 ) ) ;
#78776=DIRECTION ( 'NONE',  ( 0.000000000000000000, -0.000000000000000000, 1.000000000000000000 ) ) ;
#78777=DIRECTION ( 'NONE',  ( 0.000000000000000000, 0.000000000000000000, 1.000000000000000000 ) ) ;
#78778=AXIS2_PLACEMENT_3D ( 'NONE', #80482, #100106, #29434 ) ;
#78779=ORIENTED_EDGE ( 'NONE', *, *, #109624, .T. ) ;
#78780=EDGE_LOOP ( 'NONE', ( #104753, #5828, #13581, #40326 ) ) ;
#78781=ADVANCED_FACE ( 'NONE', ( #16489 ), #81997, .T. ) ;
#78782=ORIENTED_EDGE ( 'NONE', *, *, #34551, .T. ) ;
#78783=ORIENTED_EDGE ( 'NONE', *, *, #29173, .T. ) ;
#78784=CARTESIAN_POINT ( 'NONE',  ( 6.049999999999932321, 2.500000000000000000, -1.818653347947326138 ) ) ;
#78785=DIRECTION ( 'NONE',  ( 0.000000000000000000, 0.000000000000000000, -1.000000000000000000 ) ) ;
#78786=ORIENTED_EDGE ( 'NONE', *, *, #114728, .T. ) ;
#78787=EDGE_LOOP ( 'NONE', ( #62735, #71526, #79447, #109710 ) ) ;
#78788=VERTEX_POINT ( 'NONE', #127126 ) ;
#78790=CONICAL_SURFACE ( 'NONE', #3461, 0.09999999999999982514, 0.003490658503988666988 ) ;
#78791=CIRCLE ( 'NONE', #66237, 0.1000000000000000472 ) ;
#78792=CIRCLE ( 'NONE', #39084, 0.1000000000000002554 ) ;
#78793=DIRECTION ( 'NONE',  ( 0.000000000000000000, -0.9999939076577903929, 0.003490651415223739937 ) ) ;
#78794=PLANE ( 'NONE',  #85305 ) ;
#78795=DIRECTION ( 'NONE',  ( 0.000000000000000000, 1.000000000000000000, 0.000000000000000000 ) ) ;
#78796=CARTESIAN_POINT ( 'NONE',  ( -10.45000000000000462, 12.50000000000000000, -6.495190528383298911 ) ) ;
#78797=CARTESIAN_POINT ( 'NONE',  ( 2.500000000000002220, 1.499999999999999334, 10.00000000000000178 ) ) ;
#78798=CARTESIAN_POINT ( 'NONE',  ( -5.200000000000020606, 12.50000000000000000, -0.3464101615137782364 ) ) ;
#78799=EDGE_CURVE ( 'NONE', #112624, #76508, #94509, .T. ) ;
#78800=ORIENTED_EDGE ( 'NONE', *, *, #77017, .T. ) ;
#78801=DIRECTION ( 'NONE',  ( 0.000000000000000000, -0.000000000000000000, 1.000000000000000000 ) ) ;
#78802=ORIENTED_EDGE ( 'NONE', *, *, #44592, .T. ) ;
#78803=ORIENTED_EDGE ( 'NONE', *, *, #79469, .F. ) ;
#78804=ORIENTED_EDGE ( 'NONE', *, *, #97617, .F. ) ;
#78805=DIRECTION ( 'NONE',  ( 0.000000000000000000, -0.000000000000000000, 1.000000000000000000 ) ) ;
#78806=ORIENTED_EDGE ( 'NONE', *, *, #78158, .F. ) ;
#78807=AXIS2_PLACEMENT_3D ( 'NONE', #17401, #87440, #47538 ) ;
#78808=ORIENTED_EDGE ( 'NONE', *, *, #89273, .T. ) ;
#78809=CIRCLE ( 'NONE', #35178, 0.06509327318403745899 ) ;
#78810=CARTESIAN_POINT ( 'NONE',  ( -12.94999999999999218, 2.500000000000000000, -2.165063509461099489 ) ) ;
#78811=DIRECTION ( 'NONE',  ( 0.000000000000000000, 0.000000000000000000, -1.000000000000000000 ) ) ;
#78812=DIRECTION ( 'NONE',  ( 0.000000000000000000, -0.000000000000000000, 1.000000000000000000 ) ) ;
#78813=AXIS2_PLACEMENT_3D ( 'NONE', #28326, #39457, #38820 ) ;
#78814=DIRECTION ( 'NONE',  ( 0.000000000000000000, 0.000000000000000000, 1.000000000000000000 ) ) ;
#78815=CARTESIAN_POINT ( 'NONE',  ( -9.999999999999969802, 2.500000000000000000, 4.330127018922196314 ) ) ;
#78816=CIRCLE ( 'NONE', #122715, 0.09999999999999999167 ) ;
#78817=ORIENTED_EDGE ( 'NONE', *, *, #47795, .T. ) ;
#78818=CARTESIAN_POINT ( 'NONE',  ( -13.74999999999998934, 2.500000000000000000, -1.472243186433547901 ) ) ;
#78819=CIRCLE ( 'NONE', #59957, 0.06509327318403745899 ) ;
#78820=EDGE_LOOP ( 'NONE', ( #45246, #80142, #7944, #83049 ) ) ;
#78821=CONICAL_SURFACE ( 'NONE', #45366, 0.09999999999999982514, 0.003490658503988666988 ) ;
#78822=CARTESIAN_POINT ( 'NONE',  ( 6.449999999999931788, 12.50000000000000000, -6.148780366869526226 ) ) ;
#78823=ADVANCED_FACE ( 'NONE', ( #96344 ), #88226, .T. ) ;
#78824=ORIENTED_EDGE ( 'NONE', *, *, #39277, .F. ) ;
#78825=FACE_OUTER_BOUND ( 'NONE', #110695, .T. ) ;
#78826=DIRECTION ( 'NONE',  ( -0.000000000000000000, -1.000000000000000000, -0.000000000000000000 ) ) ;
#78827=ORIENTED_EDGE ( 'NONE', *, *, #3658, .T. ) ;
#78828=CARTESIAN_POINT ( 'NONE',  ( -8.950000000000009948, 2.500000000000000000, 2.611473670974873151 ) ) ;
#78829=CIRCLE ( 'NONE', #116447, 0.1000000000000000472 ) ;
#78830=CARTESIAN_POINT ( 'NONE',  ( 2.099999999999950351, 12.50000000000000000, -2.276824562219559311E-15 ) ) ;
#78831=ORIENTED_EDGE ( 'NONE', *, *, #52322, .T. ) ;
#78832=CONICAL_SURFACE ( 'NONE', #22388, 0.1000000000000000056, 0.003490658503988666988 ) ;
#78833=AXIS2_PLACEMENT_3D ( 'NONE', #29848, #110337, #97935 ) ;
#78834=CARTESIAN_POINT ( 'NONE',  ( -12.69999999999999218, 2.500000000000000000, -4.676537180435975216 ) ) ;
#78835=ORIENTED_EDGE ( 'NONE', *, *, #4615, .T. ) ;
#78836=ADVANCED_FACE ( 'NONE', ( #15853 ), #97004, .T. ) ;
#78837=EDGE_CURVE ( 'NONE', #6221, #87480, #38090, .T. ) ;
#78838=ORIENTED_EDGE ( 'NONE', *, *, #100222, .F. ) ;
#78839=CARTESIAN_POINT ( 'NONE',  ( -1.250000000000037970, 2.500000000000000000, 7.288010851410849256 ) ) ;
#78840=CARTESIAN_POINT ( 'NONE',  ( 3.549999999999944755, 12.50000000000000000, -6.906693963081115051 ) ) ;
#78841=ADVANCED_FACE ( 'NONE', ( #64955 ), #40154, .T. ) ;
#78843=EDGE_CURVE ( 'NONE', #102605, #118212, #76082, .T. ) ;
#78844=DIRECTION ( 'NONE',  ( 0.000000000000000000, 0.000000000000000000, -1.000000000000000000 ) ) ;
#78845=FACE_OUTER_BOUND ( 'NONE', #80072, .T. ) ;
#78846=ORIENTED_EDGE ( 'NONE', *, *, #118386, .T. ) ;
#78848=AXIS2_PLACEMENT_3D ( 'NONE', #129500, #39821, #79724 ) ;
#78849=ADVANCED_FACE ( 'NONE', ( #26987 ), #25680, .T. ) ;
#78850=ORIENTED_EDGE ( 'NONE', *, *, #8933, .F. ) ;
#78851=EDGE_CURVE ( 'NONE', #108664, #86700, #33877, .T. ) ;
#78852=PLANE ( 'NONE',  #48650 ) ;
#78853=LINE ( 'NONE', #129250, #93978 ) ;
#78854=EDGE_CURVE ( 'NONE', #33691, #86214, #25046, .T. ) ;
#78855=EDGE_LOOP ( 'NONE', ( #101405, #5731, #86222, #41323 ) ) ;
#78856=CARTESIAN_POINT ( 'NONE',  ( -3.150000000000032330, 12.50000000000000000, -6.148780366869526226 ) ) ;
#78857=CARTESIAN_POINT ( 'NONE',  ( -5.000000000000023093, 2.500000000000000000, 0.7928203230275495672 ) ) ;
#78858=DIRECTION ( 'NONE',  ( 0.000000000000000000, 1.000000000000000000, 0.000000000000000000 ) ) ;
#78859=FACE_OUTER_BOUND ( 'NONE', #68916, .T. ) ;
#78860=FACE_OUTER_BOUND ( 'NONE', #86387, .T. ) ;
#78861=ORIENTED_EDGE ( 'NONE', *, *, #17651, .T. ) ;
#78862=CARTESIAN_POINT ( 'NONE',  ( -5.200000000000022382, 2.500000000000000000, 0.4464101615137735513 ) ) ;
#78863=CIRCLE ( 'NONE', #93419, 0.06509327318403745899 ) ;
#78864=DIRECTION ( 'NONE',  ( 0.000000000000000000, 0.000000000000000000, -1.000000000000000000 ) ) ;
#78865=CARTESIAN_POINT ( 'NONE',  ( 0.3999999999999555023, 2.500000000000000000, 4.430127018922196847 ) ) ;
#78866=ORIENTED_EDGE ( 'NONE', *, *, #30447, .F. ) ;
#78867=VECTOR ( 'NONE', #43284, 1000.000000000000000 ) ;
#78868=CIRCLE ( 'NONE', #87153, 0.09999999999999999167 ) ;
#78869=CARTESIAN_POINT ( 'NONE',  ( -10.40000000000000213, 12.50000000000000000, 4.330127018922196314 ) ) ;
#78870=ORIENTED_EDGE ( 'NONE', *, *, #96543, .T. ) ;
#78871=VERTEX_POINT ( 'NONE', #85253 ) ;
#78872=FACE_OUTER_BOUND ( 'NONE', #126711, .T. ) ;
#78873=ORIENTED_EDGE ( 'NONE', *, *, #123006, .F. ) ;
#78874=CARTESIAN_POINT ( 'NONE',  ( 8.949999999999915801, 12.50000000000000000, 6.841600689897072485 ) ) ;
#78875=DIRECTION ( 'NONE',  ( 0.000000000000000000, 0.000000000000000000, 1.000000000000000000 ) ) ;
#78876=VECTOR ( 'NONE', #19406, 1000.000000000000000 ) ;
#78877=CIRCLE ( 'NONE', #60098, 0.06509327318403745899 ) ;
#78878=ORIENTED_EDGE ( 'NONE', *, *, #110786, .F. ) ;
#78879=VECTOR ( 'NONE', #89839, 1000.000000000000000 ) ;
#78880=DIRECTION ( 'NONE',  ( -0.000000000000000000, -1.000000000000000000, -0.000000000000000000 ) ) ;
#78881=DIRECTION ( 'NONE',  ( -0.000000000000000000, 1.000000000000000000, -0.000000000000000000 ) ) ;
#78882=ORIENTED_EDGE ( 'NONE', *, *, #84789, .T. ) ;
#78883=DIRECTION ( 'NONE',  ( 0.000000000000000000, 0.000000000000000000, 1.000000000000000000 ) ) ;
#78884=FACE_OUTER_BOUND ( 'NONE', #106940, .T. ) ;
#78885=ORIENTED_EDGE ( 'NONE', *, *, #24270, .T. ) ;
#78886=EDGE_CURVE ( 'NONE', #87133, #109940, #113290, .T. ) ;
#78887=VECTOR ( 'NONE', #90655, 1000.000000000000000 ) ;
#78888=ORIENTED_EDGE ( 'NONE', *, *, #64956, .T. ) ;
#78889=EDGE_CURVE ( 'NONE', #72558, #23223, #125802, .T. ) ;
#78890=ORIENTED_EDGE ( 'NONE', *, *, #25621, .T. ) ;
#78891=DIRECTION ( 'NONE',  ( 0.000000000000000000, 1.000000000000000000, 0.000000000000000000 ) ) ;
#78892=DIRECTION ( 'NONE',  ( -0.000000000000000000, 1.000000000000000000, -0.000000000000000000 ) ) ;
#78893=FACE_OUTER_BOUND ( 'NONE', #101234, .T. ) ;
#78894=FACE_BOUND ( 'NONE', #48822, .T. ) ;
#78895=ORIENTED_EDGE ( 'NONE', *, *, #16403, .F. ) ;
#78896=DIRECTION ( 'NONE',  ( -0.000000000000000000, 1.000000000000000000, -0.000000000000000000 ) ) ;
#78897=LINE ( 'NONE', #88698, #121305 ) ;
#78898=VECTOR ( 'NONE', #59405, 1000.000000000000000 ) ;
#78899=ORIENTED_EDGE ( 'NONE', *, *, #34460, .F. ) ;
#78900=EDGE_CURVE ( 'NONE', #33453, #117544, #19191, .T. ) ;
#78901=CARTESIAN_POINT ( 'NONE',  ( -3.150000000000030109, 2.500000000000000000, -2.411473670974877859 ) ) ;
#78902=CARTESIAN_POINT ( 'NONE',  ( 16.80832070733759664, 1.716026667499273239, 5.822501722867528429 ) ) ;
#78903=VECTOR ( 'NONE', #113608, 1000.000000000000000 ) ;
#78904=DIRECTION ( 'NONE',  ( 0.000000000000000000, 0.000000000000000000, 1.000000000000000000 ) ) ;
#78905=CARTESIAN_POINT ( 'NONE',  ( -7.300000000000016698, 2.500000000000000000, -0.3464101615137783474 ) ) ;
#78906=DIRECTION ( 'NONE',  ( 0.000000000000000000, 0.000000000000000000, 1.000000000000000000 ) ) ;
#78907=DIRECTION ( 'NONE',  ( 0.000000000000000000, 1.000000000000000000, 0.000000000000000000 ) ) ;
#78908=CARTESIAN_POINT ( 'NONE',  ( -12.49999999999999289, 12.50000000000000000, -4.957854068765714217 ) ) ;
#78910=AXIS2_PLACEMENT_3D ( 'NONE', #25535, #53092, #13788 ) ;
#78911=VERTEX_POINT ( 'NONE', #85 ) ;
#78912=ORIENTED_EDGE ( 'NONE', *, *, #87349, .T. ) ;
#78914=ORIENTED_EDGE ( 'NONE', *, *, #25859, .F. ) ;
#78915=VERTEX_POINT ( 'NONE', #118568 ) ;
#78916=CARTESIAN_POINT ( 'NONE',  ( -4.150000000000024336, 2.500000000000000000, -2.957883832488653830 ) ) ;
#78917=CARTESIAN_POINT ( 'NONE',  ( -1.650000000000034772, 2.500000000000000000, 6.495190528383297135 ) ) ;
#78918=AXIS2_PLACEMENT_3D ( 'NONE', #9715, #109853, #99391 ) ;
#78919=VERTEX_POINT ( 'NONE', #28269 ) ;
#78920=FACE_BOUND ( 'NONE', #82900, .T. ) ;
#78921=DIRECTION ( 'NONE',  ( 0.000000000000000000, 0.000000000000000000, -1.000000000000000000 ) ) ;
#78922=CIRCLE ( 'NONE', #53761, 0.06509327318403745899 ) ;
#78923=CIRCLE ( 'NONE', #20323, 0.06509327318403745899 ) ;
#78924=LINE ( 'NONE', #48158, #21948 ) ;
#78925=CARTESIAN_POINT ( 'NONE',  ( 6.249999999999967137, 12.50000000000000000, 6.495190528383297135 ) ) ;
#78926=DIRECTION ( 'NONE',  ( 0.000000000000000000, -0.000000000000000000, 1.000000000000000000 ) ) ;
#78927=CARTESIAN_POINT ( 'NONE',  ( 5.849999999999933920, 2.500000000000000000, 6.495190528383297135 ) ) ;
#78928=ORIENTED_EDGE ( 'NONE', *, *, #64069, .T. ) ;
#78930=EDGE_CURVE ( 'NONE', #26610, #128555, #117463, .T. ) ;
#78931=VERTEX_POINT ( 'NONE', #7969 ) ;
#78932=ORIENTED_EDGE ( 'NONE', *, *, #120786, .F. ) ;
#78933=CARTESIAN_POINT ( 'NONE',  ( -8.950000000000011724, 2.500000000000000000, -6.148780366869520897 ) ) ;
#78935=CARTESIAN_POINT ( 'NONE',  ( 2.299999999999948752, 12.50000000000000000, 0.2813168883297361700 ) ) ;
#78936=ORIENTED_EDGE ( 'NONE', *, *, #66114, .T. ) ;
#78937=LINE ( 'NONE', #29195, #7877 ) ;
#78938=DIRECTION ( 'NONE',  ( -1.000000000000000000, -0.000000000000000000, -0.000000000000000000 ) ) ;
#78939=CARTESIAN_POINT ( 'NONE',  ( -1.250000000000037526, 12.50000000000000000, -5.802370205355749988 ) ) ;
#78942=DIRECTION ( 'NONE',  ( -0.000000000000000000, 1.000000000000000000, -0.000000000000000000 ) ) ;
#78943=CARTESIAN_POINT ( 'NONE',  ( 6.049999999999932321, 2.500000000000000000, 1.818653347947321475 ) ) ;
#78944=EDGE_CURVE ( 'NONE', #29090, #81317, #410, .T. ) ;
#78945=DIRECTION ( 'NONE',  ( 0.000000000000000000, 0.000000000000000000, -1.000000000000000000 ) ) ;
#78946=EDGE_CURVE ( 'NONE', #107061, #35451, #61071, .T. ) ;
#78947=EDGE_LOOP ( 'NONE', ( #25118, #46923 ) ) ;
#78948=CARTESIAN_POINT ( 'NONE',  ( 4.349999999999941025, 12.50000000000000000, -6.148780366869526226 ) ) ;
#78949=AXIS2_PLACEMENT_3D ( 'NONE', #32602, #102588, #43067 ) ;
#78950=ORIENTED_EDGE ( 'NONE', *, *, #85320, .T. ) ;
#78951=VECTOR ( 'NONE', #53253, 1000.000000000000000 ) ;
#78952=EDGE_LOOP ( 'NONE', ( #86203, #124435, #122174, #79934 ) ) ;
#78953=CARTESIAN_POINT ( 'NONE',  ( 9.599999999999917932, 2.500000000000000000, 0.7928203230275495672 ) ) ;
#78954=DIRECTION ( 'NONE',  ( 0.000000000000000000, 0.000000000000000000, 1.000000000000000000 ) ) ;
#78955=CARTESIAN_POINT ( 'NONE',  ( -6.050000000000018474, 2.500000000000000000, 6.741600689897071952 ) ) ;
#78956=ADVANCED_FACE ( 'NONE', ( #9913 ), #59015, .T. ) ;
#78957=ORIENTED_EDGE ( 'NONE', *, *, #36344, .F. ) ;
#78958=VECTOR ( 'NONE', #126831, 1000.000000000000000 ) ;
#78959=ORIENTED_EDGE ( 'NONE', *, *, #73057, .T. ) ;
#78960=CARTESIAN_POINT ( 'NONE',  ( 9.349999999999916156, 2.500000000000000000, -1.818653347947326138 ) ) ;
#78961=AXIS2_PLACEMENT_3D ( 'NONE', #81990, #21807, #102916 ) ;
#78962=AXIS2_PLACEMENT_3D ( 'NONE', #80055, #20497, #60437 ) ;
#78963=CARTESIAN_POINT ( 'NONE',  ( -9.400000000000007461, 2.500000000000000000, -0.3464101615137783474 ) ) ;
#78964=DIRECTION ( 'NONE',  ( 0.000000000000000000, 0.000000000000000000, -1.000000000000000000 ) ) ;
#78965=ORIENTED_EDGE ( 'NONE', *, *, #18905, .F. ) ;
#78966=FACE_OUTER_BOUND ( 'NONE', #6873, .T. ) ;
#78967=ORIENTED_EDGE ( 'NONE', *, *, #45030, .F. ) ;
#78968=LINE ( 'NONE', #97942, #108444 ) ;
#78969=AXIS2_PLACEMENT_3D ( 'NONE', #88379, #128351, #56989 ) ;
#78970=ORIENTED_EDGE ( 'NONE', *, *, #75758, .F. ) ;
#78971=DIRECTION ( 'NONE',  ( 0.000000000000000000, 1.000000000000000000, 0.000000000000000000 ) ) ;
#78972=EDGE_CURVE ( 'NONE', #56832, #124839, #15005, .T. ) ;
#78973=CARTESIAN_POINT ( 'NONE',  ( 5.849999999999933031, 2.500000000000000000, 7.088010851410848190 ) ) ;
#78975=CONICAL_SURFACE ( 'NONE', #87343, 0.1000000000000002554, 0.003490658503988666988 ) ;
#78976=FACE_OUTER_BOUND ( 'NONE', #102636, .T. ) ;
#78977=VERTEX_POINT ( 'NONE', #119222 ) ;
#78978=EDGE_CURVE ( 'NONE', #90845, #57522, #98941, .T. ) ;
#78979=DIRECTION ( 'NONE',  ( 0.000000000000000000, 0.000000000000000000, 1.000000000000000000 ) ) ;
#78980=AXIS2_PLACEMENT_3D ( 'NONE', #105922, #102835, #73381 ) ;
#78981=VECTOR ( 'NONE', #116112, 1000.000000000000000 ) ;
#78982=VERTEX_POINT ( 'NONE', #19748 ) ;
#78983=ORIENTED_EDGE ( 'NONE', *, *, #2932, .T. ) ;
#78984=EDGE_CURVE ( 'NONE', #15244, #32827, #97647, .T. ) ;
#78985=ADVANCED_FACE ( 'NONE', ( #129070 ), #73575, .T. ) ;
#78986=DIRECTION ( 'NONE',  ( -4.274815082592931898E-19, -0.9999939076577903929, -0.003490651415223739937 ) ) ;
#78987=CARTESIAN_POINT ( 'NONE',  ( -4.800000000000024691, 12.50000000000000000, 4.676537180435972552 ) ) ;
#78988=CARTESIAN_POINT ( 'NONE',  ( -7.700000000000014388, 2.500000000000000000, -0.4464101615137782142 ) ) ;
#78989=EDGE_CURVE ( 'NONE', #78289, #101891, #35936, .T. ) ;
#78990=DIRECTION ( 'NONE',  ( 0.000000000000000000, -0.9999939076577903929, 0.003490651415223739937 ) ) ;
#78991=EDGE_CURVE ( 'NONE', #108881, #52645, #69376, .T. ) ;
#78992=DIRECTION ( 'NONE',  ( 0.000000000000000000, -0.9999939076577903929, 0.003490651415223739937 ) ) ;
#78993=DIRECTION ( 'NONE',  ( 0.000000000000000000, 0.000000000000000000, 1.000000000000000000 ) ) ;
#78994=CIRCLE ( 'NONE', #91589, 0.1000000000000002554 ) ;
#78995=DIRECTION ( 'NONE',  ( 0.000000000000000000, 0.000000000000000000, 1.000000000000000000 ) ) ;
#78996=PLANE ( 'NONE',  #126527 ) ;
#78997=DIRECTION ( 'NONE',  ( -0.000000000000000000, -1.000000000000000000, -0.000000000000000000 ) ) ;
#78998=EDGE_CURVE ( 'NONE', #120218, #49230, #80596, .T. ) ;
#78999=ADVANCED_FACE ( 'NONE', ( #9272 ), #4700, .T. ) ;
#79000=AXIS2_PLACEMENT_3D ( 'NONE', #48653, #171, #128529 ) ;
#79001=CIRCLE ( 'NONE', #43407, 0.1000000000000002554 ) ;
#79002=EDGE_CURVE ( 'NONE', #94563, #102844, #49218, .T. ) ;
#79003=CIRCLE ( 'NONE', #39309, 0.06509327318403745899 ) ;
#79004=EDGE_CURVE ( 'NONE', #3617, #25385, #102923, .T. ) ;
#79005=VERTEX_POINT ( 'NONE', #57738 ) ;
#79006=LINE ( 'NONE', #56734, #119455 ) ;
#79007=EDGE_CURVE ( 'NONE', #97758, #31178, #88324, .T. ) ;
#79008=FACE_OUTER_BOUND ( 'NONE', #81786, .T. ) ;
#79009=CARTESIAN_POINT ( 'NONE',  ( -13.09999999999999254, 12.50000000000000000, -4.741630453620012453 ) ) ;
#79010=PLANE ( 'NONE',  #94492 ) ;
#79011=FACE_OUTER_BOUND ( 'NONE', #123480, .T. ) ;
#79012=EDGE_CURVE ( 'NONE', #71169, #107580, #89215, .T. ) ;
#79013=ORIENTED_EDGE ( 'NONE', *, *, #50606, .F. ) ;
#79014=DIRECTION ( 'NONE',  ( 0.000000000000000000, 0.000000000000000000, 1.000000000000000000 ) ) ;
#79015=CIRCLE ( 'NONE', #14130, 0.09999999999999982514 ) ;
#79016=DIRECTION ( 'NONE',  ( 0.000000000000000000, 1.000000000000000000, 0.000000000000000000 ) ) ;
#79017=CARTESIAN_POINT ( 'NONE',  ( -1.650000000000034328, 12.50000000000000000, -6.560283801567339701 ) ) ;
#79019=ORIENTED_EDGE ( 'NONE', *, *, #101906, .F. ) ;
#79020=DIRECTION ( 'NONE',  ( -4.274815082592931898E-19, -0.9999939076577903929, -0.003490651415223739937 ) ) ;
#79021=EDGE_LOOP ( 'NONE', ( #54338, #43470, #116505, #109456 ) ) ;
#79022=VERTEX_POINT ( 'NONE', #79408 ) ;
#79023=VERTEX_POINT ( 'NONE', #119307 ) ;
#79024=CARTESIAN_POINT ( 'NONE',  ( 6.049999999999930544, 12.50000000000000000, 2.511473670974873507 ) ) ;
#79025=FACE_OUTER_BOUND ( 'NONE', #42606, .T. ) ;
#79026=DIRECTION ( 'NONE',  ( 0.000000000000000000, 1.000000000000000000, 0.000000000000000000 ) ) ;
#79027=DIRECTION ( 'NONE',  ( -0.000000000000000000, 1.000000000000000000, -0.000000000000000000 ) ) ;
#79028=ORIENTED_EDGE ( 'NONE', *, *, #123284, .T. ) ;
#79029=DIRECTION ( 'NONE',  ( 0.000000000000000000, 0.000000000000000000, -1.000000000000000000 ) ) ;
#79030=ORIENTED_EDGE ( 'NONE', *, *, #66943, .T. ) ;
#79031=DIRECTION ( 'NONE',  ( 0.000000000000000000, 0.000000000000000000, 1.000000000000000000 ) ) ;
#79032=CONICAL_SURFACE ( 'NONE', #56017, 0.1000000000000002554, 0.003490658503988666988 ) ;
#79033=DIRECTION ( 'NONE',  ( -0.000000000000000000, -1.000000000000000000, -0.000000000000000000 ) ) ;
#79034=LINE ( 'NONE', #89483, #104957 ) ;
#79035=DIRECTION ( 'NONE',  ( 0.000000000000000000, 1.000000000000000000, 0.000000000000000000 ) ) ;
#79036=ORIENTED_EDGE ( 'NONE', *, *, #120038, .F. ) ;
#79037=AXIS2_PLACEMENT_3D ( 'NONE', #122577, #1498, #2793 ) ;
#79038=EDGE_CURVE ( 'NONE', #85834, #98777, #100857, .T. ) ;
#79039=AXIS2_PLACEMENT_3D ( 'NONE', #48586, #88493, #78703 ) ;
#79040=EDGE_LOOP ( 'NONE', ( #97698, #17723, #81548, #38081 ) ) ;
#79041=VERTEX_POINT ( 'NONE', #21112 ) ;
#79042=ORIENTED_EDGE ( 'NONE', *, *, #92224, .T. ) ;
#79043=ADVANCED_FACE ( 'NONE', ( #128528 ), #90488, .T. ) ;
#79044=VERTEX_POINT ( 'NONE', #71502 ) ;
#79045=CARTESIAN_POINT ( 'NONE',  ( -5.400000000000020783, 2.500000000000000000, 5.022947341949748790 ) ) ;
#79046=DIRECTION ( 'NONE',  ( 0.000000000000000000, 1.000000000000000000, 0.000000000000000000 ) ) ;
#79047=FACE_OUTER_BOUND ( 'NONE', #4610, .T. ) ;
#79048=FACE_BOUND ( 'NONE', #56376, .T. ) ;
#79049=CARTESIAN_POINT ( 'NONE',  ( -9.150000000000009237, 12.50000000000000000, 2.230156782645134950 ) ) ;
#79051=AXIS2_PLACEMENT_3D ( 'NONE', #128789, #37594, #106949 ) ;
#79052=LINE ( 'NONE', #109114, #68580 ) ;
#79053=CARTESIAN_POINT ( 'NONE',  ( -7.900000000000014566, 2.500000000000000000, 0.6928203230275494784 ) ) ;
#79054=AXIS2_PLACEMENT_3D ( 'NONE', #77247, #27476, #67386 ) ;
#79055=DIRECTION ( 'NONE',  ( -0.000000000000000000, 1.000000000000000000, -0.000000000000000000 ) ) ;
#79056=CARTESIAN_POINT ( 'NONE',  ( -3.550000000000027800, 12.50000000000000000, 6.148780366869520009 ) ) ;
#79057=CARTESIAN_POINT ( 'NONE',  ( 1.249999999999953815, 2.500000000000000000, -2.757883832488654097 ) ) ;
#79059=DIRECTION ( 'NONE',  ( 0.000000000000000000, 1.000000000000000000, 0.000000000000000000 ) ) ;
#79060=VERTEX_POINT ( 'NONE', #19160 ) ;
#79061=ORIENTED_EDGE ( 'NONE', *, *, #125424, .F. ) ;
#79062=ORIENTED_EDGE ( 'NONE', *, *, #4777, .F. ) ;
#79063=ORIENTED_EDGE ( 'NONE', *, *, #86632, .F. ) ;
#79064=AXIS2_PLACEMENT_3D ( 'NONE', #55162, #15199, #6038 ) ;
#79065=DIRECTION ( 'NONE',  ( 0.000000000000000000, -0.9999939076577903929, 0.003490651415223739937 ) ) ;
#79066=CARTESIAN_POINT ( 'NONE',  ( 3.099999999999945022, 12.50000000000000000, -0.4115034346978157509 ) ) ;
#79067=FACE_BOUND ( 'NONE', #68283, .T. ) ;
#79068=FACE_OUTER_BOUND ( 'NONE', #93478, .T. ) ;
#79069=AXIS2_PLACEMENT_3D ( 'NONE', #54813, #83017, #14867 ) ;
#79070=( GEOMETRIC_REPRESENTATION_CONTEXT ( 3 ) GLOBAL_UNCERTAINTY_ASSIGNED_CONTEXT ( ( #25699 ) ) GLOBAL_UNIT_ASSIGNED_CONTEXT ( ( #30989, #40807, #63655 ) ) REPRESENTATION_CONTEXT ( 'NONE', 'WORKASPACE' ) );
#79071=ORIENTED_EDGE ( 'NONE', *, *, #79151, .F. ) ;
#79072=DIRECTION ( 'NONE',  ( -0.000000000000000000, 1.000000000000000000, -0.000000000000000000 ) ) ;
#79073=LINE ( 'NONE', #20788, #78720 ) ;
#79074=CARTESIAN_POINT ( 'NONE',  ( -9.150000000000009237, 12.50000000000000000, -2.922977105672691422 ) ) ;
#79075=DIRECTION ( 'NONE',  ( 0.000000000000000000, 0.000000000000000000, -1.000000000000000000 ) ) ;
#79076=LINE ( 'NONE', #10321, #80864 ) ;
#79077=CIRCLE ( 'NONE', #89523, 0.09999999999999982514 ) ;
#79078=ORIENTED_EDGE ( 'NONE', *, *, #18810, .T. ) ;
#79079=AXIS2_PLACEMENT_3D ( 'NONE', #32114, #93592, #103417 ) ;
#79080=FACE_OUTER_BOUND ( 'NONE', #62922, .T. ) ;
#79081=EDGE_CURVE ( 'NONE', #45854, #71342, #27700, .T. ) ;
#79082=VERTEX_POINT ( 'NONE', #31591 ) ;
#79083=VERTEX_POINT ( 'NONE', #69567 ) ;
#79084=DIRECTION ( 'NONE',  ( 0.000000000000000000, 0.000000000000000000, 1.000000000000000000 ) ) ;
#79085=FACE_OUTER_BOUND ( 'NONE', #107148, .T. ) ;
#79086=ORIENTED_EDGE ( 'NONE', *, *, #57580, .F. ) ;
#79087=DIRECTION ( 'NONE',  ( -0.000000000000000000, -1.000000000000000000, -0.000000000000000000 ) ) ;
#79088=CARTESIAN_POINT ( 'NONE',  ( -13.74999999999998757, 2.500000000000000000, 1.472243186433549456 ) ) ;
#79089=ORIENTED_EDGE ( 'NONE', *, *, #117956, .T. ) ;
#79090=CARTESIAN_POINT ( 'NONE',  ( -2.100000000000034284, 12.50000000000000000, -0.06509327318403980434 ) ) ;
#79092=EDGE_CURVE ( 'NONE', #51861, #47076, #111309, .T. ) ;
#79093=AXIS2_PLACEMENT_3D ( 'NONE', #88872, #7714, #28023 ) ;
#79094=ADVANCED_FACE ( 'NONE', ( #59121 ), #54893, .T. ) ;
#79095=DIRECTION ( 'NONE',  ( 0.000000000000000000, 0.000000000000000000, -1.000000000000000000 ) ) ;
#79096=ORIENTED_EDGE ( 'NONE', *, *, #40136, .T. ) ;
#79097=DIRECTION ( 'NONE',  ( 0.000000000000000000, 0.000000000000000000, 1.000000000000000000 ) ) ;
#79098=FACE_BOUND ( 'NONE', #62772, .T. ) ;
#79099=AXIS2_PLACEMENT_3D ( 'NONE', #37438, #17096, #57718 ) ;
#79100=AXIS2_PLACEMENT_3D ( 'NONE', #34766, #113953, #104134 ) ;
#79101=ORIENTED_EDGE ( 'NONE', *, *, #794, .T. ) ;
#79102=DIRECTION ( 'NONE',  ( 0.000000000000000000, 0.000000000000000000, -1.000000000000000000 ) ) ;
#79103=ORIENTED_EDGE ( 'NONE', *, *, #69950, .F. ) ;
#79107=CARTESIAN_POINT ( 'NONE',  ( 12.94999999999989981, 12.50000000000000000, -2.165063509461101710 ) ) ;
#79108=EDGE_CURVE ( 'NONE', #12415, #75136, #128068, .T. ) ;
#79109=CARTESIAN_POINT ( 'NONE',  ( 7.699999999999922018, 12.50000000000000000, 0.4115034346978109769 ) ) ;
#79110=ORIENTED_EDGE ( 'NONE', *, *, #47546, .F. ) ;
#79111=ORIENTED_EDGE ( 'NONE', *, *, #92558, .T. ) ;
#79112=ORIENTED_EDGE ( 'NONE', *, *, #84745, .T. ) ;
#79113=CARTESIAN_POINT ( 'NONE',  ( 5.799999999999934985, 2.500000000000000000, -4.430127018922202176 ) ) ;
#79114=LINE ( 'NONE', #128208, #32778 ) ;
#79115=FACE_OUTER_BOUND ( 'NONE', #83373, .T. ) ;
#79116=CIRCLE ( 'NONE', #31096, 0.1000000000000002554 ) ;
#79117=VERTEX_POINT ( 'NONE', #118666 ) ;
#79118=ORIENTED_EDGE ( 'NONE', *, *, #120501, .F. ) ;
#79119=VERTEX_POINT ( 'NONE', #40788 ) ;
#79120=CARTESIAN_POINT ( 'NONE',  ( 14.99999999999989164, 2.500000000000000000, 0.7928203230275495672 ) ) ;
#79122=AXIS2_PLACEMENT_3D ( 'NONE', #29563, #39414, #70145 ) ;
#79123=VECTOR ( 'NONE', #2984, 1000.000000000000000 ) ;
#79124=DIRECTION ( 'NONE',  ( 0.000000000000000000, -0.000000000000000000, 1.000000000000000000 ) ) ;
#79125=DIRECTION ( 'NONE',  ( 0.000000000000000000, 0.000000000000000000, 1.000000000000000000 ) ) ;
#79126=CARTESIAN_POINT ( 'NONE',  ( -10.45000000000000462, 2.500000000000000000, -6.595190528383298556 ) ) ;
#79127=DIRECTION ( 'NONE',  ( 0.000000000000000000, 1.000000000000000000, 0.000000000000000000 ) ) ;
#79128=DIRECTION ( 'NONE',  ( 0.000000000000000000, 0.000000000000000000, 1.000000000000000000 ) ) ;
#79129=FACE_OUTER_BOUND ( 'NONE', #68315, .T. ) ;
#79130=AXIS2_PLACEMENT_3D ( 'NONE', #112261, #2279, #5346 ) ;
#79131=VERTEX_POINT ( 'NONE', #101627 ) ;
#79132=CIRCLE ( 'NONE', #22697, 0.09999999999999999167 ) ;
#79134=EDGE_CURVE ( 'NONE', #26297, #1525, #30960, .T. ) ;
#79135=VECTOR ( 'NONE', #93661, 1000.000000000000000 ) ;
#79136=DIRECTION ( 'NONE',  ( 0.000000000000000000, -0.000000000000000000, 1.000000000000000000 ) ) ;
#79137=DIRECTION ( 'NONE',  ( -0.000000000000000000, -1.000000000000000000, -0.000000000000000000 ) ) ;
#79138=EDGE_LOOP ( 'NONE', ( #17134, #113833, #117488, #63872 ) ) ;
#79139=ORIENTED_EDGE ( 'NONE', *, *, #117779, .F. ) ;
#79140=EDGE_CURVE ( 'NONE', #20502, #47459, #19284, .T. ) ;
#79142=DIRECTION ( 'NONE',  ( 0.000000000000000000, 0.000000000000000000, -1.000000000000000000 ) ) ;
#79143=CARTESIAN_POINT ( 'NONE',  ( -13.74999999999995381, 12.50000000000000000, -2.165063509461099489 ) ) ;
#79144=AXIS2_PLACEMENT_3D ( 'NONE', #39550, #59170, #9416 ) ;
#79145=EDGE_CURVE ( 'NONE', #120749, #21424, #21447, .T. ) ;
#79146=CARTESIAN_POINT ( 'NONE',  ( -2.050000000000032685, 2.500000000000000000, -2.065063509461102065 ) ) ;
#79147=VECTOR ( 'NONE', #117754, 1000.000000000000000 ) ;
#79148=CARTESIAN_POINT ( 'NONE',  ( 5.849999999999932143, 2.500000000000000000, 1.572243186433545548 ) ) ;
#79149=DIRECTION ( 'NONE',  ( 0.000000000000000000, 1.000000000000000000, 0.000000000000000000 ) ) ;
#79150=LINE ( 'NONE', #68019, #85407 ) ;
#79151=EDGE_CURVE ( 'NONE', #24359, #23899, #88561, .T. ) ;
#79152=EDGE_CURVE ( 'NONE', #119576, #39789, #17212, .T. ) ;
#79153=EDGE_CURVE ( 'NONE', #89280, #54263, #31924, .T. ) ;
#79154=DIRECTION ( 'NONE',  ( 0.000000000000000000, -0.000000000000000000, 1.000000000000000000 ) ) ;
#79155=CIRCLE ( 'NONE', #20656, 0.06509327318403741736 ) ;
#79156=ORIENTED_EDGE ( 'NONE', *, *, #96712, .T. ) ;
#79157=EDGE_CURVE ( 'NONE', #34557, #24306, #46478, .T. ) ;
#79158=ORIENTED_EDGE ( 'NONE', *, *, #94242, .T. ) ;
#79160=AXIS2_PLACEMENT_3D ( 'NONE', #76728, #38097, #129078 ) ;
#79161=ORIENTED_EDGE ( 'NONE', *, *, #46171, .T. ) ;
#79162=ORIENTED_EDGE ( 'NONE', *, *, #77399, .T. ) ;
#79163=CARTESIAN_POINT ( 'NONE',  ( 4.149999999999939959, 12.50000000000000000, -2.165063509461101710 ) ) ;
#79164=DIRECTION ( 'NONE',  ( -0.000000000000000000, -1.000000000000000000, -0.000000000000000000 ) ) ;
#79165=EDGE_CURVE ( 'NONE', #13562, #3295, #33979, .T. ) ;
#79166=CONICAL_SURFACE ( 'NONE', #16418, 0.09999999999999982514, 0.003490658503988666988 ) ;
#79167=ORIENTED_EDGE ( 'NONE', *, *, #66936, .T. ) ;
#79168=CARTESIAN_POINT ( 'NONE',  ( 6.249999999999930722, 2.500000000000000000, 1.572243186433545548 ) ) ;
#79169=LINE ( 'NONE', #48400, #69603 ) ;
#79170=CARTESIAN_POINT ( 'NONE',  ( -5.800000000000022027, 12.50000000000000000, -4.330127018922201643 ) ) ;
#79171=DIRECTION ( 'NONE',  ( 0.000000000000000000, 0.000000000000000000, 1.000000000000000000 ) ) ;
#79172=VERTEX_POINT ( 'NONE', #89851 ) ;
#79173=CARTESIAN_POINT ( 'NONE',  ( -15.59999999999998010, 12.50000000000000000, -0.4115034346978133639 ) ) ;
#79174=CIRCLE ( 'NONE', #112527, 0.09999999999999982514 ) ;
#79175=CARTESIAN_POINT ( 'NONE',  ( -12.89999999999999147, 12.50000000000000000, 4.330127018922196314 ) ) ;
#79176=ORIENTED_EDGE ( 'NONE', *, *, #10662, .F. ) ;
#79177=AXIS2_PLACEMENT_3D ( 'NONE', #128291, #17667, #38632 ) ;
#79178=EDGE_LOOP ( 'NONE', ( #24730, #116588 ) ) ;
#79179=EDGE_LOOP ( 'NONE', ( #42384, #101000, #122005, #64273 ) ) ;
#79180=VERTEX_POINT ( 'NONE', #40120 ) ;
#79181=CARTESIAN_POINT ( 'NONE',  ( 3.099999999999944134, 12.50000000000000000, 4.676537180435972552 ) ) ;
#79182=FACE_OUTER_BOUND ( 'NONE', #26744, .T. ) ;
#79183=DIRECTION ( 'NONE',  ( 0.000000000000000000, 0.000000000000000000, 1.000000000000000000 ) ) ;
#79184=AXIS2_PLACEMENT_3D ( 'NONE', #26225, #123753, #104751 ) ;
#79185=VERTEX_POINT ( 'NONE', #81966 ) ;
#79186=CARTESIAN_POINT ( 'NONE',  ( 8.149999999999923972, 2.500000000000000000, 2.411473670974873862 ) ) ;
#79187=PLANE ( 'NONE',  #68416 ) ;
#79188=CONICAL_SURFACE ( 'NONE', #22854, 0.1000000000000002554, 0.003490658503988666988 ) ;
#79189=CARTESIAN_POINT ( 'NONE',  ( -2.900000000000029221, 12.50000000000000000, -2.276824562219559311E-15 ) ) ;
#79190=FACE_OUTER_BOUND ( 'NONE', #1871, .T. ) ;
#79191=ORIENTED_EDGE ( 'NONE', *, *, #72789, .T. ) ;
#79192=CONICAL_SURFACE ( 'NONE', #95901, 0.09999999999999982514, 0.003490658503988666988 ) ;
#79193=CIRCLE ( 'NONE', #77030, 0.06509327318403745899 ) ;
#79194=FACE_OUTER_BOUND ( 'NONE', #23821, .T. ) ;
#79195=ADVANCED_FACE ( 'NONE', ( #23056 ), #36030, .T. ) ;
#79196=ORIENTED_EDGE ( 'NONE', *, *, #127785, .F. ) ;
#79197=ORIENTED_EDGE ( 'NONE', *, *, #55022, .F. ) ;
#79198=FACE_OUTER_BOUND ( 'NONE', #80714, .T. ) ;
#79199=DIRECTION ( 'NONE',  ( 0.000000000000000000, 0.000000000000000000, -1.000000000000000000 ) ) ;
#79200=FACE_BOUND ( 'NONE', #128131, .T. ) ;
#79201=CARTESIAN_POINT ( 'NONE',  ( 9.999999999999912959, 2.500000000000000000, 3.737306695894644371 ) ) ;
#79202=CARTESIAN_POINT ( 'NONE',  ( 14.99999999999989342, 12.50000000000000000, -0.6928203230275541413 ) ) ;
#79203=DIRECTION ( 'NONE',  ( 0.000000000000000000, 0.000000000000000000, 1.000000000000000000 ) ) ;
#79204=EDGE_CURVE ( 'NONE', #87232, #55744, #2554, .T. ) ;
#79205=VERTEX_POINT ( 'NONE', #3412 ) ;
#79206=CARTESIAN_POINT ( 'NONE',  ( -4.800000000000028244, 12.50000000000000000, -3.983716857408426293 ) ) ;
#79207=DIRECTION ( 'NONE',  ( -0.000000000000000000, 1.000000000000000000, -0.000000000000000000 ) ) ;
#79208=DIRECTION ( 'NONE',  ( -0.000000000000000000, 1.000000000000000000, -0.000000000000000000 ) ) ;
#79210=VERTEX_POINT ( 'NONE', #84550 ) ;
#79211=CARTESIAN_POINT ( 'NONE',  ( 0.3999999999999628852, 2.500000000000000000, -0.6928203230275520319 ) ) ;
#79212=AXIS2_PLACEMENT_3D ( 'NONE', #20542, #60483, #4556 ) ;
#79213=FACE_OUTER_BOUND ( 'NONE', #104002, .T. ) ;
#79214=VERTEX_POINT ( 'NONE', #64895 ) ;
#79215=ORIENTED_EDGE ( 'NONE', *, *, #92306, .T. ) ;
#79216=DIRECTION ( 'NONE',  ( 0.000000000000000000, 0.000000000000000000, -1.000000000000000000 ) ) ;
#79217=CARTESIAN_POINT ( 'NONE',  ( -9.200000000000006395, 2.500000000000000000, 4.430127018922196847 ) ) ;
#79218=FACE_BOUND ( 'NONE', #4373, .T. ) ;
#79219=DIRECTION ( 'NONE',  ( 0.000000000000000000, 0.000000000000000000, -1.000000000000000000 ) ) ;
#79220=CIRCLE ( 'NONE', #58388, 0.06509327318403745899 ) ;
#79221=AXIS2_PLACEMENT_3D ( 'NONE', #113891, #44495, #54957 ) ;
#79222=VECTOR ( 'NONE', #126771, 1000.000000000000000 ) ;
#79223=DIRECTION ( 'NONE',  ( -0.000000000000000000, -1.000000000000000000, -0.000000000000000000 ) ) ;
#79224=ORIENTED_EDGE ( 'NONE', *, *, #38630, .F. ) ;
#79225=CARTESIAN_POINT ( 'NONE',  ( 5.599999999999934808, 12.50000000000000000, -4.741630453620016006 ) ) ;
#79227=AXIS2_PLACEMENT_3D ( 'NONE', #98492, #88692, #38985 ) ;
#79228=ORIENTED_EDGE ( 'NONE', *, *, #110861, .F. ) ;
#79229=DIRECTION ( 'NONE',  ( -0.000000000000000000, -1.000000000000000000, -0.000000000000000000 ) ) ;
#79230=DIRECTION ( 'NONE',  ( 0.000000000000000000, 0.000000000000000000, 1.000000000000000000 ) ) ;
#79231=AXIS2_PLACEMENT_3D ( 'NONE', #29410, #9759, #49704 ) ;
#79232=ADVANCED_FACE ( 'NONE', ( #42056 ), #96644, .T. ) ;
#79233=DIRECTION ( 'NONE',  ( 0.000000000000000000, 1.000000000000000000, 0.000000000000000000 ) ) ;
#79234=CARTESIAN_POINT ( 'NONE',  ( 8.549999999999920774, 2.500000000000000000, 6.148780366869520897 ) ) ;
#79235=AXIS2_PLACEMENT_3D ( 'NONE', #4848, #26450, #42381 ) ;
#79236=ADVANCED_FACE ( 'NONE', ( #72806 ), #94595, .T. ) ;
#79237=ORIENTED_EDGE ( 'NONE', *, *, #129164, .T. ) ;
#79238=CARTESIAN_POINT ( 'NONE',  ( 3.149999999999942624, 2.500000000000000000, 6.148780366869520897 ) ) ;
#79239=FACE_OUTER_BOUND ( 'NONE', #57745, .T. ) ;
#79240=CARTESIAN_POINT ( 'NONE',  ( -12.94999999999999218, 12.50000000000000000, 2.099970236277064028 ) ) ;
#79241=AXIS2_PLACEMENT_3D ( 'NONE', #64654, #36507, #26029 ) ;
#79242=CARTESIAN_POINT ( 'NONE',  ( -9.150000000000009237, 2.500000000000000000, -1.572243186433550211 ) ) ;
#79243=VERTEX_POINT ( 'NONE', #23700 ) ;
#79244=ADVANCED_FACE ( 'NONE', ( #54436 ), #82086, .T. ) ;
#79245=ORIENTED_EDGE ( 'NONE', *, *, #27421, .F. ) ;
#79246=EDGE_CURVE ( 'NONE', #40987, #18162, #115517, .T. ) ;
#79247=CARTESIAN_POINT ( 'NONE',  ( 2.499999999999948930, 12.50000000000000000, -5.022947341949754119 ) ) ;
#79248=ORIENTED_EDGE ( 'NONE', *, *, #60685, .T. ) ;
#79249=CARTESIAN_POINT ( 'NONE',  ( 6.649999999999930189, 2.500000000000000000, 5.902370205355745192 ) ) ;
#79250=CARTESIAN_POINT ( 'NONE',  ( 17.50000000000000000, -2.499999999999999556, -0.6666666666666614116 ) ) ;
#79251=CARTESIAN_POINT ( 'NONE',  ( -8.100000000000013856, 2.500000000000000000, -3.983716857408426293 ) ) ;
#79252=DIRECTION ( 'NONE',  ( -0.000000000000000000, -1.000000000000000000, -0.000000000000000000 ) ) ;
#79253=ORIENTED_EDGE ( 'NONE', *, *, #41783, .T. ) ;
#79254=AXIS2_PLACEMENT_3D ( 'NONE', #114233, #6190, #5552 ) ;
#79255=ADVANCED_FACE ( 'NONE', ( #13216 ), #15165, .T. ) ;
#79256=CARTESIAN_POINT ( 'NONE',  ( 9.349999999999916156, 12.50000000000000000, -2.511473670974877948 ) ) ;
#79257=DIRECTION ( 'NONE',  ( 0.000000000000000000, 0.000000000000000000, 1.000000000000000000 ) ) ;
#79258=DIRECTION ( 'NONE',  ( -0.000000000000000000, 1.000000000000000000, -0.000000000000000000 ) ) ;
#79260=CARTESIAN_POINT ( 'NONE',  ( 8.749999999999923617, 2.500000000000000000, 1.572243186433545548 ) ) ;
#79261=EDGE_CURVE ( 'NONE', #25034, #35273, #73668, .T. ) ;
#79262=CONICAL_SURFACE ( 'NONE', #110543, 0.1000000000000002554, 0.003490658503988666988 ) ;
#79263=LINE ( 'NONE', #126419, #118355 ) ;
#79264=AXIS2_PLACEMENT_3D ( 'NONE', #10433, #40567, #50359 ) ;
#79266=EDGE_LOOP ( 'NONE', ( #23585, #67998 ) ) ;
#79267=FACE_OUTER_BOUND ( 'NONE', #105586, .T. ) ;
#79268=ORIENTED_EDGE ( 'NONE', *, *, #6872, .F. ) ;
#79269=CARTESIAN_POINT ( 'NONE',  ( -0.8500000000000382805, 12.50000000000000000, -5.737276932171712751 ) ) ;
#79270=ORIENTED_EDGE ( 'NONE', *, *, #42028, .T. ) ;
#79271=ORIENTED_EDGE ( 'NONE', *, *, #127694, .F. ) ;
#79272=EDGE_LOOP ( 'NONE', ( #105068, #51605, #123445, #83156 ) ) ;
#79273=AXIS2_PLACEMENT_3D ( 'NONE', #120144, #91322, #347 ) ;
#79274=DIRECTION ( 'NONE',  ( 0.000000000000000000, -0.000000000000000000, 1.000000000000000000 ) ) ;
#79275=DIRECTION ( 'NONE',  ( 0.000000000000000000, 0.000000000000000000, 1.000000000000000000 ) ) ;
#79276=CARTESIAN_POINT ( 'NONE',  ( -10.20000000000000284, 12.50000000000000000, -0.2813168883297408329 ) ) ;
#79278=AXIS2_PLACEMENT_3D ( 'NONE', #56114, #81867, #35846 ) ;
#79279=VECTOR ( 'NONE', #81133, 1000.000000000000000 ) ;
#79280=LINE ( 'NONE', #30831, #13816 ) ;
#79281=DIRECTION ( 'NONE',  ( 0.000000000000000000, 0.000000000000000000, 1.000000000000000000 ) ) ;
#79282=LINE ( 'NONE', #110025, #83605 ) ;
#79284=DIRECTION ( 'NONE',  ( -4.274815082592931898E-19, -0.9999939076577903929, -0.003490651415223739937 ) ) ;
#79285=AXIS2_PLACEMENT_3D ( 'NONE', #111583, #51396, #79551 ) ;
#79286=CARTESIAN_POINT ( 'NONE',  ( -1.850000000000033840, 2.500000000000000000, 2.511473670974873507 ) ) ;
#79287=ORIENTED_EDGE ( 'NONE', *, *, #72768, .F. ) ;
#79288=AXIS2_PLACEMENT_3D ( 'NONE', #31974, #62077, #111139 ) ;
#79289=CIRCLE ( 'NONE', #60511, 0.06509327318403745899 ) ;
#79290=ORIENTED_EDGE ( 'NONE', *, *, #105449, .T. ) ;
#79291=FACE_OUTER_BOUND ( 'NONE', #93935, .T. ) ;
#79292=ORIENTED_EDGE ( 'NONE', *, *, #2939, .F. ) ;
#79293=EDGE_LOOP ( 'NONE', ( #44242, #107599 ) ) ;
#79294=DIRECTION ( 'NONE',  ( 0.000000000000000000, 1.000000000000000000, 0.000000000000000000 ) ) ;
#79295=EDGE_CURVE ( 'NONE', #112355, #7480, #71619, .T. ) ;
#79296=DIRECTION ( 'NONE',  ( 0.000000000000000000, 1.000000000000000000, 0.000000000000000000 ) ) ;
#79297=PLANE ( 'NONE',  #61116 ) ;
#79298=CARTESIAN_POINT ( 'NONE',  ( -5.850000000000021849, 2.500000000000000000, -2.757883832488654097 ) ) ;
#79299=EDGE_CURVE ( 'NONE', #94406, #120997, #505, .T. ) ;
#79300=CARTESIAN_POINT ( 'NONE',  ( 0.4499999999999569344, 12.50000000000000000, 2.165063509461097713 ) ) ;
#79301=AXIS2_PLACEMENT_3D ( 'NONE', #12717, #112876, #13374 ) ;
#79302=ORIENTED_EDGE ( 'NONE', *, *, #94886, .T. ) ;
#79303=ADVANCED_FACE ( 'NONE', ( #12573 ), #113388, .T. ) ;
#79304=EDGE_CURVE ( 'NONE', #21644, #38111, #69465, .T. ) ;
#79305=ADVANCED_FACE ( 'NONE', ( #34174 ), #77978, .T. ) ;
#79306=ORIENTED_EDGE ( 'NONE', *, *, #16186, .T. ) ;
#79307=AXIS2_PLACEMENT_3D ( 'NONE', #83039, #72571, #122317 ) ;
#79308=DIRECTION ( 'NONE',  ( 0.000000000000000000, 0.000000000000000000, 1.000000000000000000 ) ) ;
#79309=AXIS2_PLACEMENT_3D ( 'NONE', #127593, #68665, #69296 ) ;
#79310=VERTEX_POINT ( 'NONE', #114019 ) ;
#79311=FACE_OUTER_BOUND ( 'NONE', #92578, .T. ) ;
#79312=ADVANCED_FACE ( 'NONE', ( #24350 ), #64259, .T. ) ;
#79313=EDGE_LOOP ( 'NONE', ( #93474, #10112, #23911, #55293 ) ) ;
#79314=ORIENTED_EDGE ( 'NONE', *, *, #73819, .F. ) ;
#79315=CARTESIAN_POINT ( 'NONE',  ( 3.349999999999941913, 12.50000000000000000, 6.495190528383297135 ) ) ;
#79316=AXIS2_PLACEMENT_3D ( 'NONE', #74163, #114084, #14575 ) ;
#79317=DIRECTION ( 'NONE',  ( 0.000000000000000000, -0.000000000000000000, 1.000000000000000000 ) ) ;
#79318=AXIS2_PLACEMENT_3D ( 'NONE', #38413, #78335, #108411 ) ;
#79319=EDGE_CURVE ( 'NONE', #47762, #46559, #111410, .T. ) ;
#79320=AXIS2_PLACEMENT_3D ( 'NONE', #65568, #97606, #106770 ) ;
#79321=ADVANCED_FACE ( 'NONE', ( #2108 ), #82632, .T. ) ;
#79322=DIRECTION ( 'NONE',  ( 0.000000000000000000, 0.000000000000000000, -1.000000000000000000 ) ) ;
#79323=CARTESIAN_POINT ( 'NONE',  ( -10.65000000000000213, 2.500000000000000000, 1.818653347947321475 ) ) ;
#79324=DIRECTION ( 'NONE',  ( 0.000000000000000000, 0.000000000000000000, 1.000000000000000000 ) ) ;
#79325=ORIENTED_EDGE ( 'NONE', *, *, #107208, .F. ) ;
#79326=DIRECTION ( 'NONE',  ( 0.000000000000000000, 0.000000000000000000, 1.000000000000000000 ) ) ;
#79327=CARTESIAN_POINT ( 'NONE',  ( 2.699999999999946443, 2.500000000000000000, 0.2464101615137735679 ) ) ;
#79328=DIRECTION ( 'NONE',  ( 0.000000000000000000, 1.000000000000000000, 0.000000000000000000 ) ) ;
#79329=DIRECTION ( 'NONE',  ( 0.000000000000000000, 0.000000000000000000, 1.000000000000000000 ) ) ;
#79330=AXIS2_PLACEMENT_3D ( 'NONE', #78072, #68244, #58449 ) ;
#79331=DIRECTION ( 'NONE',  ( -0.000000000000000000, -1.000000000000000000, -0.000000000000000000 ) ) ;
#79332=AXIS2_PLACEMENT_3D ( 'NONE', #910, #50042, #9451 ) ;
#79333=ORIENTED_EDGE ( 'NONE', *, *, #44271, .T. ) ;
#79334=CONICAL_SURFACE ( 'NONE', #85570, 0.1000000000000000472, 0.003490658503988666988 ) ;
#79335=ORIENTED_EDGE ( 'NONE', *, *, #47488, .F. ) ;
#79336=PLANE ( 'NONE',  #119788 ) ;
#79337=EDGE_LOOP ( 'NONE', ( #62804, #70960, #94603, #122049 ) ) ;
#79338=DIRECTION ( 'NONE',  ( -0.000000000000000000, -1.000000000000000000, -0.000000000000000000 ) ) ;
#79339=DIRECTION ( 'NONE',  ( -0.000000000000000000, -1.000000000000000000, -0.000000000000000000 ) ) ;
#79340=CIRCLE ( 'NONE', #106415, 0.1000000000000002554 ) ;
#79341=ORIENTED_EDGE ( 'NONE', *, *, #28157, .F. ) ;
#79342=DIRECTION ( 'NONE',  ( -4.274815082592931898E-19, -0.9999939076577903929, -0.003490651415223739937 ) ) ;
#79343=CARTESIAN_POINT ( 'NONE',  ( -3.350000000000028955, 2.500000000000000000, 5.702370205355745014 ) ) ;
#79345=CARTESIAN_POINT ( 'NONE',  ( 5.399999999999934630, 12.50000000000000000, -0.6928203230275542523 ) ) ;
#79346=ORIENTED_EDGE ( 'NONE', *, *, #125521, .T. ) ;
#79347=DIRECTION ( 'NONE',  ( -0.000000000000000000, 1.000000000000000000, -0.000000000000000000 ) ) ;
#79348=EDGE_LOOP ( 'NONE', ( #46837, #52467 ) ) ;
#79349=DIRECTION ( 'NONE',  ( 0.000000000000000000, 1.000000000000000000, 0.000000000000000000 ) ) ;
#79350=AXIS2_PLACEMENT_3D ( 'NONE', #102310, #12615, #95064 ) ;
#79352=DIRECTION ( 'NONE',  ( 0.000000000000000000, 1.000000000000000000, 0.000000000000000000 ) ) ;
#79353=ADVANCED_FACE ( 'NONE', ( #117195 ), #5334, .T. ) ;
#79354=VERTEX_POINT ( 'NONE', #107409 ) ;
#79355=CARTESIAN_POINT ( 'NONE',  ( 6.649999999999931966, 12.50000000000000000, -5.737276932171712751 ) ) ;
#79356=ORIENTED_EDGE ( 'NONE', *, *, #26816, .F. ) ;
#79357=FACE_OUTER_BOUND ( 'NONE', #113178, .T. ) ;
#79358=AXIS2_PLACEMENT_3D ( 'NONE', #49983, #194, #80065 ) ;
#79359=FACE_OUTER_BOUND ( 'NONE', #125735, .T. ) ;
#79360=DIRECTION ( 'NONE',  ( 0.000000000000000000, 0.000000000000000000, 1.000000000000000000 ) ) ;
#79361=VERTEX_POINT ( 'NONE', #115263 ) ;
#79362=DIRECTION ( 'NONE',  ( 0.000000000000000000, 0.000000000000000000, -1.000000000000000000 ) ) ;
#79363=CIRCLE ( 'NONE', #56352, 0.1000000000000002554 ) ;
#79364=CIRCLE ( 'NONE', #98123, 0.06509327318403741736 ) ;
#79365=DIRECTION ( 'NONE',  ( -4.274815082592931898E-19, -0.9999939076577903929, -0.003490651415223739937 ) ) ;
#79366=ORIENTED_EDGE ( 'NONE', *, *, #29814, .T. ) ;
#79367=DIRECTION ( 'NONE',  ( -0.000000000000000000, -1.000000000000000000, -0.000000000000000000 ) ) ;
#79369=DIRECTION ( 'NONE',  ( -0.000000000000000000, -1.000000000000000000, -0.000000000000000000 ) ) ;
#79370=CIRCLE ( 'NONE', #54233, 0.06509327318403745899 ) ;
#79371=CIRCLE ( 'NONE', #22938, 0.06509327318403745899 ) ;
#79372=ORIENTED_EDGE ( 'NONE', *, *, #65791, .T. ) ;
#79373=CARTESIAN_POINT ( 'NONE',  ( 4.399999999999937295, 2.500000000000000000, 4.776537180435972196 ) ) ;
#79374=CARTESIAN_POINT ( 'NONE',  ( 10.04522989427052160, 2.499999999999999112, -8.164691043833789408 ) ) ;
#79375=EDGE_LOOP ( 'NONE', ( #108147, #94111 ) ) ;
#79376=ORIENTED_EDGE ( 'NONE', *, *, #108672, .F. ) ;
#79377=PLANE ( 'NONE',  #33141 ) ;
#79378=DIRECTION ( 'NONE',  ( -0.000000000000000000, 1.000000000000000000, -0.000000000000000000 ) ) ;
#79379=EDGE_LOOP ( 'NONE', ( #20005, #105734, #59640, #6189 ) ) ;
#79380=CARTESIAN_POINT ( 'NONE',  ( 3.949999999999942446, 2.500000000000000000, -6.941600689897078347 ) ) ;
#79382=DIRECTION ( 'NONE',  ( 0.000000000000000000, 0.000000000000000000, 1.000000000000000000 ) ) ;
#79384=CARTESIAN_POINT ( 'NONE',  ( -11.05000000000000071, 2.500000000000000000, 2.511473670974873507 ) ) ;
#79385=CARTESIAN_POINT ( 'NONE',  ( -4.150000000000024336, 2.500000000000000000, -2.165063509461101710 ) ) ;
#79386=DIRECTION ( 'NONE',  ( 0.000000000000000000, -0.9999939076577903929, 0.003490651415223739937 ) ) ;
#79387=CIRCLE ( 'NONE', #31368, 0.09999999999999982514 ) ;
#79388=ADVANCED_FACE ( 'NONE', ( #35463 ), #92545, .T. ) ;
#79389=CIRCLE ( 'NONE', #93961, 0.1000000000000000472 ) ;
#79390=ORIENTED_EDGE ( 'NONE', *, *, #41288, .F. ) ;
#79391=ORIENTED_EDGE ( 'NONE', *, *, #21171, .F. ) ;
#79392=VERTEX_POINT ( 'NONE', #55731 ) ;
#79393=ORIENTED_EDGE ( 'NONE', *, *, #106874, .T. ) ;
#79394=CARTESIAN_POINT ( 'NONE',  ( 1.649999999999951505, 2.500000000000000000, -1.472243186433550122 ) ) ;
#79395=DIRECTION ( 'NONE',  ( -0.000000000000000000, 1.000000000000000000, -0.000000000000000000 ) ) ;
#79396=DIRECTION ( 'NONE',  ( 0.000000000000000000, 0.000000000000000000, 1.000000000000000000 ) ) ;
#79397=ORIENTED_EDGE ( 'NONE', *, *, #97344, .F. ) ;
#79398=EDGE_CURVE ( 'NONE', #76857, #32813, #25739, .T. ) ;
#79399=FACE_BOUND ( 'NONE', #96938, .T. ) ;
#79400=ORIENTED_EDGE ( 'NONE', *, *, #108724, .F. ) ;
#79401=EDGE_CURVE ( 'NONE', #85979, #58087, #23596, .T. ) ;
#79402=CARTESIAN_POINT ( 'NONE',  ( 14.14999999999989555, 2.500000000000000000, 2.265063509461097357 ) ) ;
#79403=DIRECTION ( 'NONE',  ( 0.000000000000000000, 1.000000000000000000, 0.000000000000000000 ) ) ;
#79404=AXIS2_PLACEMENT_3D ( 'NONE', #72715, #51154, #21687 ) ;
#79405=AXIS2_PLACEMENT_3D ( 'NONE', #114223, #14061, #74944 ) ;
#79406=DIRECTION ( 'NONE',  ( 0.000000000000000000, 1.000000000000000000, 0.000000000000000000 ) ) ;
#79407=CARTESIAN_POINT ( 'NONE',  ( 7.049999999999930544, 12.50000000000000000, -6.495190528383302464 ) ) ;
#79408=CARTESIAN_POINT ( 'NONE',  ( 9.999999999999911182, 2.500000000000000000, -3.537306695894649966 ) ) ;
#79409=EDGE_CURVE ( 'NONE', #81872, #34821, #127690, .T. ) ;
#79410=FACE_OUTER_BOUND ( 'NONE', #53380, .T. ) ;
#79411=EDGE_CURVE ( 'NONE', #40041, #26625, #87119, .T. ) ;
#79412=FACE_OUTER_BOUND ( 'NONE', #7463, .T. ) ;
#79413=DIRECTION ( 'NONE',  ( 0.000000000000000000, 0.000000000000000000, -1.000000000000000000 ) ) ;
#79414=EDGE_CURVE ( 'NONE', #56250, #42358, #15796, .T. ) ;
#79415=DIRECTION ( 'NONE',  ( 0.000000000000000000, 1.000000000000000000, 0.000000000000000000 ) ) ;
#79416=ADVANCED_FACE ( 'NONE', ( #117859 ), #42491, .T. ) ;
#79417=CONICAL_SURFACE ( 'NONE', #60551, 0.1000000000000002554, 0.003490658503988666988 ) ;
#79418=PLANE ( 'NONE',  #12553 ) ;
#79419=CIRCLE ( 'NONE', #37647, 0.1000000000000000472 ) ;
#79420=EDGE_LOOP ( 'NONE', ( #51840, #48212, #124102, #25603 ) ) ;
#79421=VERTEX_POINT ( 'NONE', #15138 ) ;
#79422=VECTOR ( 'NONE', #71440, 1000.000000000000000 ) ;
#79423=ORIENTED_EDGE ( 'NONE', *, *, #73250, .T. ) ;
#79424=ORIENTED_EDGE ( 'NONE', *, *, #8893, .T. ) ;
#79425=DIRECTION ( 'NONE',  ( -0.000000000000000000, -1.000000000000000000, -0.000000000000000000 ) ) ;
#79426=CARTESIAN_POINT ( 'NONE',  ( 1.849999999999950129, 2.500000000000000000, -6.741600689897078169 ) ) ;
#79427=ORIENTED_EDGE ( 'NONE', *, *, #58566, .T. ) ;
#79428=ORIENTED_EDGE ( 'NONE', *, *, #62386, .T. ) ;
#79429=EDGE_CURVE ( 'NONE', #34708, #78443, #29865, .T. ) ;
#79430=ORIENTED_EDGE ( 'NONE', *, *, #60576, .T. ) ;
#79431=DIRECTION ( 'NONE',  ( 0.000000000000000000, 0.000000000000000000, 1.000000000000000000 ) ) ;
#79432=CARTESIAN_POINT ( 'NONE',  ( -5.200000000000020606, 2.500000000000000000, -0.3464101615137782364 ) ) ;
#79433=CARTESIAN_POINT ( 'NONE',  ( 13.74999999999989342, 2.500000000000000000, -1.472243186433550122 ) ) ;
#79434=CARTESIAN_POINT ( 'NONE',  ( -14.14999999999998792, 2.500000000000000000, -1.472243186433547901 ) ) ;
#79435=DIRECTION ( 'NONE',  ( -0.000000000000000000, -1.000000000000000000, -0.000000000000000000 ) ) ;
#79436=CIRCLE ( 'NONE', #89782, 0.06509327318403741736 ) ;
#79437=CARTESIAN_POINT ( 'NONE',  ( 7.499999999999925393, 12.50000000000000000, -3.572213422710612374 ) ) ;
#79438=FACE_OUTER_BOUND ( 'NONE', #55895, .T. ) ;
#79439=VERTEX_POINT ( 'NONE', #76016 ) ;
#79440=FACE_OUTER_BOUND ( 'NONE', #84983, .T. ) ;
#79441=EDGE_LOOP ( 'NONE', ( #7063, #11349, #29293, #17017 ) ) ;
#79442=ORIENTED_EDGE ( 'NONE', *, *, #123260, .T. ) ;
#79443=ORIENTED_EDGE ( 'NONE', *, *, #10165, .F. ) ;
#79444=DIRECTION ( 'NONE',  ( 0.000000000000000000, -0.000000000000000000, 1.000000000000000000 ) ) ;
#79445=EDGE_CURVE ( 'NONE', #101675, #20773, #105158, .T. ) ;
#79446=EDGE_LOOP ( 'NONE', ( #86882, #23949 ) ) ;
#79447=ORIENTED_EDGE ( 'NONE', *, *, #27416, .T. ) ;
#79448=DIRECTION ( 'NONE',  ( -0.000000000000000000, -1.000000000000000000, -0.000000000000000000 ) ) ;
#79449=DIRECTION ( 'NONE',  ( 0.000000000000000000, 0.000000000000000000, 1.000000000000000000 ) ) ;
#79450=CARTESIAN_POINT ( 'NONE',  ( 13.09999999999990195, 2.500000000000000000, -3.883716857408426648 ) ) ;
#79451=DIRECTION ( 'NONE',  ( 0.000000000000000000, 0.000000000000000000, 1.000000000000000000 ) ) ;
#79452=EDGE_CURVE ( 'NONE', #75136, #12415, #71719, .T. ) ;
#79453=CIRCLE ( 'NONE', #41811, 0.1000000000000000472 ) ;
#79454=VERTEX_POINT ( 'NONE', #45282 ) ;
#79455=ADVANCED_FACE ( 'NONE', ( #95660 ), #85192, .T. ) ;
#79456=CARTESIAN_POINT ( 'NONE',  ( 11.24999999999990763, 12.50000000000000000, 1.407149913249508000 ) ) ;
#79457=ORIENTED_EDGE ( 'NONE', *, *, #114599, .T. ) ;
#79458=CARTESIAN_POINT ( 'NONE',  ( 8.099999999999923261, 2.500000000000000000, -3.983716857408426293 ) ) ;
#79459=ADVANCED_FACE ( 'NONE', ( #6591 ), #45930, .T. ) ;
#79460=AXIS2_PLACEMENT_3D ( 'NONE', #67052, #106989, #7507 ) ;
#79461=VERTEX_POINT ( 'NONE', #115939 ) ;
#79462=DIRECTION ( 'NONE',  ( 0.000000000000000000, 0.000000000000000000, -1.000000000000000000 ) ) ;
#79463=DIRECTION ( 'NONE',  ( 0.000000000000000000, 0.000000000000000000, 1.000000000000000000 ) ) ;
#79464=ORIENTED_EDGE ( 'NONE', *, *, #53214, .F. ) ;
#79465=CARTESIAN_POINT ( 'NONE',  ( -0.6000000000000388356, 12.50000000000000000, 4.611443907251934426 ) ) ;
#79466=EDGE_CURVE ( 'NONE', #81575, #46684, #37395, .T. ) ;
#79467=DIRECTION ( 'NONE',  ( 0.000000000000000000, 0.000000000000000000, 1.000000000000000000 ) ) ;
#79468=VERTEX_POINT ( 'NONE', #106123 ) ;
#79469=EDGE_CURVE ( 'NONE', #62361, #2581, #76668, .T. ) ;
#79470=CIRCLE ( 'NONE', #66915, 0.09999999999999982514 ) ;
#79471=CIRCLE ( 'NONE', #114942, 0.06509327318403745899 ) ;
#79472=EDGE_CURVE ( 'NONE', #113011, #104247, #38281, .T. ) ;
#79473=EDGE_CURVE ( 'NONE', #26951, #76450, #59222, .T. ) ;
#79474=DIRECTION ( 'NONE',  ( 0.000000000000000000, 0.000000000000000000, -1.000000000000000000 ) ) ;
#79475=EDGE_LOOP ( 'NONE', ( #30331, #73440, #97752, #18553 ) ) ;
#79476=ORIENTED_EDGE ( 'NONE', *, *, #58817, .F. ) ;
#79477=DIRECTION ( 'NONE',  ( -0.000000000000000000, -1.000000000000000000, -0.000000000000000000 ) ) ;
#79478=FACE_OUTER_BOUND ( 'NONE', #40398, .T. ) ;
#79480=DIRECTION ( 'NONE',  ( 0.000000000000000000, 0.000000000000000000, -1.000000000000000000 ) ) ;
#79482=CARTESIAN_POINT ( 'NONE',  ( -10.20000000000000462, 12.50000000000000000, 4.676537180435972552 ) ) ;
#79483=ORIENTED_EDGE ( 'NONE', *, *, #5238, .F. ) ;
#79485=ORIENTED_EDGE ( 'NONE', *, *, #85932, .T. ) ;
#79486=CARTESIAN_POINT ( 'NONE',  ( -10.00000000000000355, 2.500000000000000000, -0.6928203230275541413 ) ) ;
#79487=CIRCLE ( 'NONE', #64873, 0.09999999999999982514 ) ;
#79488=CARTESIAN_POINT ( 'NONE',  ( 14.14999999999989555, 12.50000000000000000, 2.165063509461097713 ) ) ;
#79489=VECTOR ( 'NONE', #83436, 1000.000000000000000 ) ;
#79490=DIRECTION ( 'NONE',  ( -0.000000000000000000, 1.000000000000000000, -0.000000000000000000 ) ) ;
#79491=DIRECTION ( 'NONE',  ( -0.000000000000000000, -1.000000000000000000, -0.000000000000000000 ) ) ;
#79492=DIRECTION ( 'NONE',  ( 0.000000000000000000, 1.000000000000000000, 0.000000000000000000 ) ) ;
#79493=CARTESIAN_POINT ( 'NONE',  ( -9.800000000000007816, 12.50000000000000000, -4.048810130592459089 ) ) ;
#79495=ORIENTED_EDGE ( 'NONE', *, *, #106467, .T. ) ;
#79496=AXIS2_PLACEMENT_3D ( 'NONE', #30091, #102038, #122332 ) ;
#79497=DIRECTION ( 'NONE',  ( 0.000000000000000000, 0.000000000000000000, 1.000000000000000000 ) ) ;
#79498=CARTESIAN_POINT ( 'NONE',  ( 0.4499999999999573785, 2.500000000000000000, -6.495190528383302464 ) ) ;
#79499=AXIS2_PLACEMENT_3D ( 'NONE', #10310, #66155, #39791 ) ;
#79500=ORIENTED_EDGE ( 'NONE', *, *, #7734, .F. ) ;
#79501=CARTESIAN_POINT ( 'NONE',  ( -0.4500000000000402012, 2.500000000000000000, 2.265063509461097357 ) ) ;
#79502=AXIS2_PLACEMENT_3D ( 'NONE', #20405, #50496, #49880 ) ;
#79503=AXIS2_PLACEMENT_3D ( 'NONE', #124266, #34616, #16213 ) ;
#79504=EDGE_CURVE ( 'NONE', #18510, #79117, #48748, .T. ) ;
#79505=EDGE_LOOP ( 'NONE', ( #22875, #119578, #28383, #79965 ) ) ;
#79506=VERTEX_POINT ( 'NONE', #49798 ) ;
#79507=DIRECTION ( 'NONE',  ( 0.000000000000000000, -0.000000000000000000, 1.000000000000000000 ) ) ;
#79508=EDGE_LOOP ( 'NONE', ( #105326, #94530 ) ) ;
#79509=CARTESIAN_POINT ( 'NONE',  ( -0.2000000000000339284, 2.500000000000000000, -0.3464101615137759604 ) ) ;
#79510=DIRECTION ( 'NONE',  ( -0.000000000000000000, 1.000000000000000000, -0.000000000000000000 ) ) ;
#79511=CIRCLE ( 'NONE', #16777, 0.09999999999999999167 ) ;
#79512=ORIENTED_EDGE ( 'NONE', *, *, #96396, .F. ) ;
#79513=PLANE ( 'NONE',  #126102 ) ;
#79514=DIRECTION ( 'NONE',  ( 0.000000000000000000, 0.000000000000000000, 1.000000000000000000 ) ) ;
#79515=EDGE_LOOP ( 'NONE', ( #104559, #29759 ) ) ;
#79516=CONICAL_SURFACE ( 'NONE', #123330, 0.09999999999999999167, 0.003490658503988666988 ) ;
#79517=DIRECTION ( 'NONE',  ( -0.000000000000000000, 1.000000000000000000, -0.000000000000000000 ) ) ;
#79518=EDGE_CURVE ( 'NONE', #16084, #64702, #2757, .T. ) ;
#79519=ORIENTED_EDGE ( 'NONE', *, *, #43829, .F. ) ;
#79520=ORIENTED_EDGE ( 'NONE', *, *, #114551, .T. ) ;
#79521=ORIENTED_EDGE ( 'NONE', *, *, #7006, .T. ) ;
#79522=LINE ( 'NONE', #61165, #39980 ) ;
#79523=CARTESIAN_POINT ( 'NONE',  ( 7.899999999999924860, 2.500000000000000000, -3.537306695894649966 ) ) ;
#79524=CARTESIAN_POINT ( 'NONE',  ( -14.14999999999998614, 2.500000000000000000, 1.372243186433549367 ) ) ;
#79525=FACE_BOUND ( 'NONE', #3834, .T. ) ;
#79526=EDGE_LOOP ( 'NONE', ( #45535, #44241 ) ) ;
#79527=DIRECTION ( 'NONE',  ( -0.000000000000000000, 1.000000000000000000, -0.000000000000000000 ) ) ;
#79528=DIRECTION ( 'NONE',  ( 0.000000000000000000, -0.9999939076577903929, 0.003490651415223739937 ) ) ;
#79529=ORIENTED_EDGE ( 'NONE', *, *, #116388, .T. ) ;
#79530=CARTESIAN_POINT ( 'NONE',  ( -2.300000000000033129, 2.500000000000000000, 3.983716857408420076 ) ) ;
#79531=DIRECTION ( 'NONE',  ( -0.000000000000000000, -1.000000000000000000, -0.000000000000000000 ) ) ;
#79532=VECTOR ( 'NONE', #99247, 1000.000000000000000 ) ;
#79533=DIRECTION ( 'NONE',  ( -0.000000000000000000, -1.000000000000000000, -0.000000000000000000 ) ) ;
#79534=CARTESIAN_POINT ( 'NONE',  ( -14.59999999999998366, 12.50000000000000000, 0.6928203230275518099 ) ) ;
#79535=CARTESIAN_POINT ( 'NONE',  ( -0.8000000000000381251, 2.500000000000000000, 4.430127018922196847 ) ) ;
#79536=CONICAL_SURFACE ( 'NONE', #54385, 0.1000000000000002554, 0.003490658503988666988 ) ;
#79537=DIRECTION ( 'NONE',  ( -0.000000000000000000, -1.000000000000000000, -0.000000000000000000 ) ) ;
#79538=DIRECTION ( 'NONE',  ( 0.000000000000000000, 0.000000000000000000, -1.000000000000000000 ) ) ;
#79539=EDGE_CURVE ( 'NONE', #36792, #28566, #107220, .T. ) ;
#79540=CONICAL_SURFACE ( 'NONE', #41896, 0.09999999999999982514, 0.003490658503988666988 ) ;
#79541=VERTEX_POINT ( 'NONE', #10485 ) ;
#79542=ORIENTED_EDGE ( 'NONE', *, *, #126095, .F. ) ;
#79543=ORIENTED_EDGE ( 'NONE', *, *, #2182, .T. ) ;
#79545=ORIENTED_EDGE ( 'NONE', *, *, #98371, .F. ) ;
#79546=DIRECTION ( 'NONE',  ( -0.000000000000000000, -1.000000000000000000, -0.000000000000000000 ) ) ;
#79547=PLANE ( 'NONE',  #94814 ) ;
#79548=VERTEX_POINT ( 'NONE', #69405 ) ;
#79549=FACE_BOUND ( 'NONE', #114452, .T. ) ;
#79550=ADVANCED_FACE ( 'NONE', ( #79881 ), #125989, .T. ) ;
#79551=DIRECTION ( 'NONE',  ( 0.000000000000000000, 0.000000000000000000, 1.000000000000000000 ) ) ;
#79552=DIRECTION ( 'NONE',  ( -0.000000000000000000, -1.000000000000000000, -0.000000000000000000 ) ) ;
#79553=DIRECTION ( 'NONE',  ( 0.000000000000000000, 0.000000000000000000, 1.000000000000000000 ) ) ;
#79554=EDGE_CURVE ( 'NONE', #53683, #58504, #39968, .T. ) ;
#79555=DIRECTION ( 'NONE',  ( 0.000000000000000000, -0.9999939076577903929, 0.003490651415223739937 ) ) ;
#79556=EDGE_CURVE ( 'NONE', #23819, #126044, #13113, .T. ) ;
#79557=DIRECTION ( 'NONE',  ( 0.000000000000000000, 0.000000000000000000, -1.000000000000000000 ) ) ;
#79558=EDGE_CURVE ( 'NONE', #112102, #11681, #98905, .T. ) ;
#79559=DIRECTION ( 'NONE',  ( -0.000000000000000000, -1.000000000000000000, -0.000000000000000000 ) ) ;
#79560=ADVANCED_FACE ( 'NONE', ( #109992 ), #15252, .T. ) ;
#79561=ORIENTED_EDGE ( 'NONE', *, *, #42842, .F. ) ;
#79562=EDGE_CURVE ( 'NONE', #21250, #127872, #118511, .T. ) ;
#79563=ORIENTED_EDGE ( 'NONE', *, *, #121855, .F. ) ;
#79564=ORIENTED_EDGE ( 'NONE', *, *, #36687, .T. ) ;
#79565=ORIENTED_EDGE ( 'NONE', *, *, #26434, .T. ) ;
#79566=ORIENTED_EDGE ( 'NONE', *, *, #63590, .T. ) ;
#79567=CARTESIAN_POINT ( 'NONE',  ( 15.83209681635554666, 2.500000000000000000, 5.404881881984142211 ) ) ;
#79568=DIRECTION ( 'NONE',  ( -0.000000000000000000, -1.000000000000000000, -0.000000000000000000 ) ) ;
#79569=VERTEX_POINT ( 'NONE', #49157 ) ;
#79570=EDGE_CURVE ( 'NONE', #72840, #120418, #86275, .T. ) ;
#79571=DIRECTION ( 'NONE',  ( 0.000000000000000000, 1.000000000000000000, 0.000000000000000000 ) ) ;
#79572=EDGE_CURVE ( 'NONE', #90854, #127558, #119806, .T. ) ;
#79573=FACE_OUTER_BOUND ( 'NONE', #325, .T. ) ;
#79574=ADVANCED_FACE ( 'NONE', ( #30804 ), #100955, .T. ) ;
#79575=DIRECTION ( 'NONE',  ( 0.000000000000000000, 1.000000000000000000, 0.000000000000000000 ) ) ;
#79577=CARTESIAN_POINT ( 'NONE',  ( 3.549999999999944755, 2.500000000000000000, -2.611473670974877592 ) ) ;
#79578=DIRECTION ( 'NONE',  ( 0.000000000000000000, 1.000000000000000000, 0.000000000000000000 ) ) ;
#79579=DIRECTION ( 'NONE',  ( -0.000000000000000000, 1.000000000000000000, -0.000000000000000000 ) ) ;
#79580=ORIENTED_EDGE ( 'NONE', *, *, #27273, .T. ) ;
#79581=DIRECTION ( 'NONE',  ( -0.000000000000000000, 1.000000000000000000, -0.000000000000000000 ) ) ;
#79582=CIRCLE ( 'NONE', #12657, 0.06509327318403745899 ) ;
#79583=ORIENTED_EDGE ( 'NONE', *, *, #126850, .T. ) ;
#79584=ORIENTED_EDGE ( 'NONE', *, *, #112206, .T. ) ;
#79585=DIRECTION ( 'NONE',  ( 0.000000000000000000, 0.000000000000000000, -1.000000000000000000 ) ) ;
#79586=DIRECTION ( 'NONE',  ( 0.000000000000000000, -0.9999939076577903929, 0.003490651415223739937 ) ) ;
#79587=CARTESIAN_POINT ( 'NONE',  ( 1.249999999999953815, 2.500000000000000000, -2.857883832488653741 ) ) ;
#79588=ORIENTED_EDGE ( 'NONE', *, *, #79845, .F. ) ;
#79589=ORIENTED_EDGE ( 'NONE', *, *, #111682, .F. ) ;
#79591=CIRCLE ( 'NONE', #75464, 0.06509327318403745899 ) ;
#79593=FACE_OUTER_BOUND ( 'NONE', #83183, .T. ) ;
#79594=DIRECTION ( 'NONE',  ( 0.000000000000000000, 1.000000000000000000, 0.000000000000000000 ) ) ;
#79595=EDGE_LOOP ( 'NONE', ( #109028, #79837 ) ) ;
#79596=DIRECTION ( 'NONE',  ( 0.000000000000000000, 0.000000000000000000, -1.000000000000000000 ) ) ;
#79597=AXIS2_PLACEMENT_3D ( 'NONE', #16215, #56152, #6383 ) ;
#79598=VERTEX_POINT ( 'NONE', #39344 ) ;
#79599=DIRECTION ( 'NONE',  ( 0.000000000000000000, -0.9999939076577903929, 0.003490651415223739937 ) ) ;
#79600=EDGE_LOOP ( 'NONE', ( #15077, #79521, #111724, #92499 ) ) ;
#79601=CARTESIAN_POINT ( 'NONE',  ( -7.050000000000016698, 12.50000000000000000, -2.165063509461101710 ) ) ;
#79602=DIRECTION ( 'NONE',  ( 0.000000000000000000, -0.000000000000000000, 1.000000000000000000 ) ) ;
#79603=AXIS2_PLACEMENT_3D ( 'NONE', #92909, #57317, #125409 ) ;
#79605=EDGE_CURVE ( 'NONE', #113972, #51049, #670, .T. ) ;
#79606=DIRECTION ( 'NONE',  ( -0.000000000000000000, 1.000000000000000000, -0.000000000000000000 ) ) ;
#79607=VERTEX_POINT ( 'NONE', #40632 ) ;
#79608=ADVANCED_FACE ( 'NONE', ( #70706 ), #82189, .T. ) ;
#79609=DIRECTION ( 'NONE',  ( -0.000000000000000000, 1.000000000000000000, -0.000000000000000000 ) ) ;
#79610=EDGE_CURVE ( 'NONE', #63429, #5496, #9010, .T. ) ;
#79611=ORIENTED_EDGE ( 'NONE', *, *, #8320, .T. ) ;
#79612=ORIENTED_EDGE ( 'NONE', *, *, #43362, .F. ) ;
#79613=CARTESIAN_POINT ( 'NONE',  ( 14.14999999999989733, 12.50000000000000000, 1.472243186433545459 ) ) ;
#79614=CARTESIAN_POINT ( 'NONE',  ( 7.949999999999925571, 2.500000000000000000, 2.265063509461097357 ) ) ;
#79615=FACE_OUTER_BOUND ( 'NONE', #3327, .T. ) ;
#79616=DIRECTION ( 'NONE',  ( -0.000000000000000000, 1.000000000000000000, -0.000000000000000000 ) ) ;
#79617=EDGE_CURVE ( 'NONE', #48600, #77665, #36332, .T. ) ;
#79618=CARTESIAN_POINT ( 'NONE',  ( 2.899999999999944844, 2.500000000000000000, 5.022947341949748790 ) ) ;
#79619=CARTESIAN_POINT ( 'NONE',  ( 5.449999999999937117, 2.500000000000000000, -6.495190528383302464 ) ) ;
#79620=FACE_OUTER_BOUND ( 'NONE', #43524, .T. ) ;
#79621=DIRECTION ( 'NONE',  ( 0.000000000000000000, 0.000000000000000000, 1.000000000000000000 ) ) ;
#79622=AXIS2_PLACEMENT_3D ( 'NONE', #3608, #125945, #105682 ) ;
#79623=CIRCLE ( 'NONE', #90071, 0.1000000000000002554 ) ;
#79624=VECTOR ( 'NONE', #52703, 1000.000000000000000 ) ;
#79625=VECTOR ( 'NONE', #121182, 1000.000000000000000 ) ;
#79626=ORIENTED_EDGE ( 'NONE', *, *, #58600, .F. ) ;
#79627=LINE ( 'NONE', #50820, #14973 ) ;
#79628=DIRECTION ( 'NONE',  ( 0.000000000000000000, 0.000000000000000000, 1.000000000000000000 ) ) ;
#79629=DIRECTION ( 'NONE',  ( 0.000000000000000000, 0.000000000000000000, -1.000000000000000000 ) ) ;
#79630=EDGE_CURVE ( 'NONE', #55154, #26833, #72008, .T. ) ;
#79631=DIRECTION ( 'NONE',  ( 0.000000000000000000, 1.000000000000000000, 0.000000000000000000 ) ) ;
#79632=CARTESIAN_POINT ( 'NONE',  ( -2.950000000000030376, 2.500000000000000000, 6.395190528383296602 ) ) ;
#79633=VERTEX_POINT ( 'NONE', #101461 ) ;
#79634=DIRECTION ( 'NONE',  ( 0.000000000000000000, 0.000000000000000000, -1.000000000000000000 ) ) ;
#79635=DIRECTION ( 'NONE',  ( -4.274815082592931898E-19, -0.9999939076577903929, -0.003490651415223739937 ) ) ;
#79636=DIRECTION ( 'NONE',  ( 0.000000000000000000, 0.000000000000000000, 1.000000000000000000 ) ) ;
#79637=EDGE_LOOP ( 'NONE', ( #84492, #8456, #17370, #41965 ) ) ;
#79638=ORIENTED_EDGE ( 'NONE', *, *, #78576, .F. ) ;
#79639=CARTESIAN_POINT ( 'NONE',  ( -5.650000000000019895, 2.500000000000000000, 6.148780366869520009 ) ) ;
#79640=VECTOR ( 'NONE', #114492, 1000.000000000000000 ) ;
#79641=EDGE_CURVE ( 'NONE', #91540, #1964, #2855, .T. ) ;
#79642=VERTEX_POINT ( 'NONE', #82476 ) ;
#79643=VERTEX_POINT ( 'NONE', #105150 ) ;
#79644=ORIENTED_EDGE ( 'NONE', *, *, #92897, .T. ) ;
#79645=CARTESIAN_POINT ( 'NONE',  ( -4.800000000000024691, 2.500000000000000000, 4.776537180435972196 ) ) ;
#79646=DIRECTION ( 'NONE',  ( -0.000000000000000000, 1.000000000000000000, -0.000000000000000000 ) ) ;
#79647=DIRECTION ( 'NONE',  ( 0.000000000000000000, 0.000000000000000000, 1.000000000000000000 ) ) ;
#79648=CARTESIAN_POINT ( 'NONE',  ( 7.499999999999923617, 2.500000000000000000, 0.6928203230275494784 ) ) ;
#79649=AXIS2_PLACEMENT_3D ( 'NONE', #54984, #113263, #54343 ) ;
#79650=VERTEX_POINT ( 'NONE', #114964 ) ;
#79651=CIRCLE ( 'NONE', #77677, 0.06509327318403745899 ) ;
#79652=B_SPLINE_CURVE_WITH_KNOTS ( 'NONE', 3,
 ( #117346, #85970, #67625, #8068 ),
 .UNSPECIFIED., .F., .F.,
 ( 4, 4 ),
 ( 0.0001556283592076939662, 0.002283789722394891780 ),
 .UNSPECIFIED. ) ;
#79653=CARTESIAN_POINT ( 'NONE',  ( 14.79999999999989235, 2.500000000000000000, 0.3464101615137735735 ) ) ;
#79654=ORIENTED_EDGE ( 'NONE', *, *, #189, .F. ) ;
#79655=DIRECTION ( 'NONE',  ( 0.000000000000000000, 1.000000000000000000, 0.000000000000000000 ) ) ;
#79656=CARTESIAN_POINT ( 'NONE',  ( 18.78720903128151321, 2.539625591034162078, 4.564429507519030871 ) ) ;
#79657=DIRECTION ( 'NONE',  ( -0.000000000000000000, -1.000000000000000000, -0.000000000000000000 ) ) ;
#79658=EDGE_CURVE ( 'NONE', #24306, #34557, #78067, .T. ) ;
#79659=CARTESIAN_POINT ( 'NONE',  ( 12.09999999999990550, 2.500000000000000000, 4.330127018922196314 ) ) ;
#79660=VECTOR ( 'NONE', #99736, 1000.000000000000000 ) ;
#79661=ORIENTED_EDGE ( 'NONE', *, *, #96861, .F. ) ;
#79662=CIRCLE ( 'NONE', #19007, 0.1000000000000002554 ) ;
#79663=VERTEX_POINT ( 'NONE', #5653 ) ;
#79664=ORIENTED_EDGE ( 'NONE', *, *, #93171, .T. ) ;
#79665=EDGE_LOOP ( 'NONE', ( #44119, #9352 ) ) ;
#79666=VERTEX_POINT ( 'NONE', #2590 ) ;
#79667=DIRECTION ( 'NONE',  ( -0.000000000000000000, 1.000000000000000000, -0.000000000000000000 ) ) ;
#79668=CARTESIAN_POINT ( 'NONE',  ( -5.650000000000023448, 2.500000000000000000, -6.048780366869526581 ) ) ;
#79669=EDGE_CURVE ( 'NONE', #41193, #64688, #81803, .T. ) ;
#79670=FACE_OUTER_BOUND ( 'NONE', #90620, .T. ) ;
#79671=FACE_BOUND ( 'NONE', #75373, .T. ) ;
#79672=DIRECTION ( 'NONE',  ( 0.000000000000000000, -0.9999939076577903929, 0.003490651415223739937 ) ) ;
#79674=DIRECTION ( 'NONE',  ( 0.000000000000000000, 1.000000000000000000, 0.000000000000000000 ) ) ;
#79675=CONICAL_SURFACE ( 'NONE', #81812, 0.09999999999999982514, 0.003490658503988666988 ) ;
#79676=AXIS2_PLACEMENT_3D ( 'NONE', #57951, #129289, #46845 ) ;
#79677=PLANE ( 'NONE',  #17158 ) ;
#79678=DIRECTION ( 'NONE',  ( 0.000000000000000000, 0.000000000000000000, 1.000000000000000000 ) ) ;
#79679=CARTESIAN_POINT ( 'NONE',  ( 11.89999999999990798, 12.50000000000000000, 3.983716857408420964 ) ) ;
#79680=CIRCLE ( 'NONE', #25377, 0.06509327318403745899 ) ;
#79681=CARTESIAN_POINT ( 'NONE',  ( -8.750000000000010658, 12.50000000000000000, -1.472243186433550122 ) ) ;
#79682=ADVANCED_FACE ( 'NONE', ( #44965 ), #92266, .T. ) ;
#79683=ORIENTED_EDGE ( 'NONE', *, *, #2530, .F. ) ;
#79684=AXIS2_PLACEMENT_3D ( 'NONE', #57966, #40263, #30456 ) ;
#79685=ORIENTED_EDGE ( 'NONE', *, *, #39223, .F. ) ;
#79686=EDGE_LOOP ( 'NONE', ( #124654, #41345 ) ) ;
#79687=ORIENTED_EDGE ( 'NONE', *, *, #7339, .T. ) ;
#79688=DIRECTION ( 'NONE',  ( 0.000000000000000000, 0.000000000000000000, 1.000000000000000000 ) ) ;
#79689=CARTESIAN_POINT ( 'NONE',  ( 5.799999999999933209, 12.50000000000000000, 0.06509327318403504425 ) ) ;
#79690=FACE_BOUND ( 'NONE', #73325, .T. ) ;
#79691=DIRECTION ( 'NONE',  ( 0.000000000000000000, 0.000000000000000000, 1.000000000000000000 ) ) ;
#79693=VERTEX_POINT ( 'NONE', #105810 ) ;
#79694=ADVANCED_FACE ( 'NONE', ( #115611 ), #19583, .T. ) ;
#79695=LINE ( 'NONE', #99353, #50941 ) ;
#79696=CARTESIAN_POINT ( 'NONE',  ( -9.400000000000007461, 2.500000000000000000, 4.676537180435972552 ) ) ;
#79697=EDGE_CURVE ( 'NONE', #60583, #19106, #117756, .T. ) ;
#79698=CARTESIAN_POINT ( 'NONE',  ( 10.39999999999991509, 2.500000000000000000, 0.6928203230275494784 ) ) ;
#79699=EDGE_CURVE ( 'NONE', #87317, #107669, #96839, .T. ) ;
#79700=CARTESIAN_POINT ( 'NONE',  ( 11.24999999999990585, 2.500000000000000000, -5.802370205355749988 ) ) ;
#79701=ADVANCED_FACE ( 'NONE', ( #56047 ), #95347, .T. ) ;
#79702=VERTEX_POINT ( 'NONE', #25291 ) ;
#79703=LINE ( 'NONE', #29976, #76395 ) ;
#79704=ORIENTED_EDGE ( 'NONE', *, *, #113737, .F. ) ;
#79705=ADVANCED_FACE ( 'NONE', ( #22273 ), #103111, .T. ) ;
#79706=AXIS2_PLACEMENT_3D ( 'NONE', #36643, #66070, #54963 ) ;
#79707=EDGE_LOOP ( 'NONE', ( #110565, #36977 ) ) ;
#79708=CIRCLE ( 'NONE', #37949, 0.06509327318403745899 ) ;
#79709=DIRECTION ( 'NONE',  ( 0.000000000000000000, 1.000000000000000000, 0.000000000000000000 ) ) ;
#79710=AXIS2_PLACEMENT_3D ( 'NONE', #36309, #97788, #76865 ) ;
#79711=EDGE_CURVE ( 'NONE', #102673, #120910, #113583, .T. ) ;
#79712=CARTESIAN_POINT ( 'NONE',  ( 3.549999999999943867, 12.50000000000000000, -1.818653347947326138 ) ) ;
#79713=ORIENTED_EDGE ( 'NONE', *, *, #59194, .F. ) ;
#79714=EDGE_CURVE ( 'NONE', #9888, #41869, #701, .T. ) ;
#79715=EDGE_CURVE ( 'NONE', #39357, #77678, #9113, .T. ) ;
#79716=FACE_OUTER_BOUND ( 'NONE', #69758, .T. ) ;
#79717=AXIS2_PLACEMENT_3D ( 'NONE', #53093, #123737, #14430 ) ;
#79718=EDGE_CURVE ( 'NONE', #92091, #29934, #111247, .T. ) ;
#79719=DIRECTION ( 'NONE',  ( -0.000000000000000000, -1.000000000000000000, -0.000000000000000000 ) ) ;
#79720=VERTEX_POINT ( 'NONE', #94689 ) ;
#79721=DIRECTION ( 'NONE',  ( -0.000000000000000000, 1.000000000000000000, -0.000000000000000000 ) ) ;
#79722=VERTEX_POINT ( 'NONE', #86140 ) ;
#79723=CIRCLE ( 'NONE', #8595, 0.06509327318403745899 ) ;
#79724=DIRECTION ( 'NONE',  ( 0.000000000000000000, 0.000000000000000000, 1.000000000000000000 ) ) ;
#79725=EDGE_CURVE ( 'NONE', #11513, #36138, #38385, .T. ) ;
#79726=VERTEX_POINT ( 'NONE', #106449 ) ;
#79727=CARTESIAN_POINT ( 'NONE',  ( 13.74999999999993427, 12.50000000000000000, 2.165063509461097713 ) ) ;
#79728=FACE_BOUND ( 'NONE', #113547, .T. ) ;
#79729=VERTEX_POINT ( 'NONE', #108382 ) ;
#79730=LINE ( 'NONE', #67294, #1589 ) ;
#79731=VERTEX_POINT ( 'NONE', #37718 ) ;
#79732=DIRECTION ( 'NONE',  ( -0.000000000000000000, 1.000000000000000000, -0.000000000000000000 ) ) ;
#79733=DIRECTION ( 'NONE',  ( 0.000000000000000000, -0.9999939076577903929, 0.003490651415223739937 ) ) ;
#79734=DIRECTION ( 'NONE',  ( -0.000000000000000000, -1.000000000000000000, -0.000000000000000000 ) ) ;
#79735=CARTESIAN_POINT ( 'NONE',  ( 2.299999999999948752, 12.50000000000000000, -3.983716857408426293 ) ) ;
#79736=DIRECTION ( 'NONE',  ( 0.000000000000000000, 1.000000000000000000, 0.000000000000000000 ) ) ;
#79737=ORIENTED_EDGE ( 'NONE', *, *, #79711, .F. ) ;
#79738=VERTEX_POINT ( 'NONE', #98542 ) ;
#79739=VERTEX_POINT ( 'NONE', #7598 ) ;
#79740=DIRECTION ( 'NONE',  ( -0.000000000000000000, 1.000000000000000000, -0.000000000000000000 ) ) ;
#79741=CARTESIAN_POINT ( 'NONE',  ( 14.39999999999989555, 12.50000000000000000, 0.3464101615137736845 ) ) ;
#79742=DIRECTION ( 'NONE',  ( -4.274815082592931898E-19, -0.9999939076577903929, -0.003490651415223739937 ) ) ;
#79743=ORIENTED_EDGE ( 'NONE', *, *, #93980, .T. ) ;
#79744=ORIENTED_EDGE ( 'NONE', *, *, #7568, .T. ) ;
#79745=ORIENTED_EDGE ( 'NONE', *, *, #30810, .F. ) ;
#79746=CARTESIAN_POINT ( 'NONE',  ( 12.49999999999990585, 12.50000000000000000, 3.637306695894644726 ) ) ;
#79747=CIRCLE ( 'NONE', #90190, 0.09999999999999982514 ) ;
#79748=EDGE_LOOP ( 'NONE', ( #1143, #41263 ) ) ;
#79749=DIRECTION ( 'NONE',  ( 0.000000000000000000, 1.000000000000000000, 0.000000000000000000 ) ) ;
#79750=AXIS2_PLACEMENT_3D ( 'NONE', #56565, #76233, #6173 ) ;
#79751=CARTESIAN_POINT ( 'NONE',  ( -3.950000000000024603, 2.500000000000000000, -2.611473670974877592 ) ) ;
#79752=DIRECTION ( 'NONE',  ( 0.000000000000000000, 1.000000000000000000, 0.000000000000000000 ) ) ;
#79753=CARTESIAN_POINT ( 'NONE',  ( -0.4000000000000331624, 2.500000000000000000, 0.000000000000000000 ) ) ;
#79754=CARTESIAN_POINT ( 'NONE',  ( 6.649999999999931966, 2.500000000000000000, -5.902370205355750521 ) ) ;
#79755=CARTESIAN_POINT ( 'NONE',  ( 12.49999999999993605, 12.50000000000000000, -0.06509327318403970719 ) ) ;
#79756=DIRECTION ( 'NONE',  ( 0.000000000000000000, 1.000000000000000000, 0.000000000000000000 ) ) ;
#79757=AXIS2_PLACEMENT_3D ( 'NONE', #118443, #102043, #71277 ) ;
#79759=AXIS2_PLACEMENT_3D ( 'NONE', #6476, #27432, #115823 ) ;
#79760=ORIENTED_EDGE ( 'NONE', *, *, #1476, .T. ) ;
#79761=EDGE_CURVE ( 'NONE', #119463, #98563, #59319, .T. ) ;
#79762=DIRECTION ( 'NONE',  ( 0.000000000000000000, 1.000000000000000000, 0.000000000000000000 ) ) ;
#79764=ORIENTED_EDGE ( 'NONE', *, *, #11403, .F. ) ;
#79765=ORIENTED_EDGE ( 'NONE', *, *, #20288, .T. ) ;
#79767=DIRECTION ( 'NONE',  ( -4.274815082592931898E-19, -0.9999939076577903929, -0.003490651415223739937 ) ) ;
#79768=LINE ( 'NONE', #81070, #26953 ) ;
#79769=CONICAL_SURFACE ( 'NONE', #327, 0.09999999999999999167, 0.003490658503988666988 ) ;
#79770=ADVANCED_FACE ( 'NONE', ( #18060 ), #37080, .T. ) ;
#79771=DIRECTION ( 'NONE',  ( -0.000000000000000000, -1.000000000000000000, -0.000000000000000000 ) ) ;
#79773=AXIS2_PLACEMENT_3D ( 'NONE', #103011, #63093, #65004 ) ;
#79774=CARTESIAN_POINT ( 'NONE',  ( -2.950000000000029932, 12.50000000000000000, 2.099970236277060032 ) ) ;
#79775=DIRECTION ( 'NONE',  ( 0.000000000000000000, 0.000000000000000000, 1.000000000000000000 ) ) ;
#79776=AXIS2_PLACEMENT_3D ( 'NONE', #122787, #52124, #33134 ) ;
#79777=DIRECTION ( 'NONE',  ( 0.000000000000000000, 1.000000000000000000, 0.000000000000000000 ) ) ;
#79778=AXIS2_PLACEMENT_3D ( 'NONE', #31711, #12686, #60548 ) ;
#79779=CARTESIAN_POINT ( 'NONE',  ( 12.09999999999990195, 2.500000000000000000, -2.276824562219559311E-15 ) ) ;
#79780=ORIENTED_EDGE ( 'NONE', *, *, #83449, .T. ) ;
#79781=AXIS2_PLACEMENT_3D ( 'NONE', #121873, #83254, #72143 ) ;
#79782=CONICAL_SURFACE ( 'NONE', #73511, 0.09999999999999982514, 0.003490658503988666988 ) ;
#79783=ORIENTED_EDGE ( 'NONE', *, *, #30562, .T. ) ;
#79784=ORIENTED_EDGE ( 'NONE', *, *, #13126, .T. ) ;
#79785=ORIENTED_EDGE ( 'NONE', *, *, #46005, .F. ) ;
#79786=CARTESIAN_POINT ( 'NONE',  ( 5.199999999999935341, 2.500000000000000000, -0.4464101615137783252 ) ) ;
#79787=DIRECTION ( 'NONE',  ( 0.000000000000000000, 0.000000000000000000, 1.000000000000000000 ) ) ;
#79788=ORIENTED_EDGE ( 'NONE', *, *, #6555, .F. ) ;
#79789=DIRECTION ( 'NONE',  ( -0.000000000000000000, 1.000000000000000000, -0.000000000000000000 ) ) ;
#79790=CARTESIAN_POINT ( 'NONE',  ( 3.749999999999978684, 12.50000000000000000, -6.560283801567339701 ) ) ;
#79791=CARTESIAN_POINT ( 'NONE',  ( 10.84999999999991260, 2.500000000000000000, 6.495190528383297135 ) ) ;
#79792=CARTESIAN_POINT ( 'NONE',  ( -5.000000000000022204, 2.500000000000000000, 3.537306695894645081 ) ) ;
#79793=ORIENTED_EDGE ( 'NONE', *, *, #44260, .T. ) ;
#79794=DIRECTION ( 'NONE',  ( 0.000000000000000000, 0.000000000000000000, 1.000000000000000000 ) ) ;
#79795=DIRECTION ( 'NONE',  ( 0.000000000000000000, -0.9999939076577903929, 0.003490651415223739937 ) ) ;
#79796=ADVANCED_FACE ( 'NONE', ( #49489 ), #44624, .T. ) ;
#79797=EDGE_LOOP ( 'NONE', ( #63349, #49608, #25024, #61805 ) ) ;
#79798=ORIENTED_EDGE ( 'NONE', *, *, #118086, .F. ) ;
#79799=ORIENTED_EDGE ( 'NONE', *, *, #15607, .T. ) ;
#79800=AXIS2_PLACEMENT_3D ( 'NONE', #6535, #28813, #108644 ) ;
#79801=VERTEX_POINT ( 'NONE', #67811 ) ;
#79802=DIRECTION ( 'NONE',  ( 0.000000000000000000, -0.9999939076577903929, 0.003490651415223739937 ) ) ;
#79803=AXIS2_PLACEMENT_3D ( 'NONE', #100372, #110193, #71543 ) ;
#79805=FACE_OUTER_BOUND ( 'NONE', #31950, .T. ) ;
#79806=VECTOR ( 'NONE', #71946, 1000.000000000000000 ) ;
#79807=AXIS2_PLACEMENT_3D ( 'NONE', #41606, #30502, #70401 ) ;
#79808=EDGE_CURVE ( 'NONE', #88035, #110508, #107741, .T. ) ;
#79809=ORIENTED_EDGE ( 'NONE', *, *, #120201, .T. ) ;
#79810=DIRECTION ( 'NONE',  ( 0.000000000000000000, 1.000000000000000000, 0.000000000000000000 ) ) ;
#79811=CARTESIAN_POINT ( 'NONE',  ( 6.849999999999927702, 2.500000000000000000, 2.411473670974873862 ) ) ;
#79812=AXIS2_PLACEMENT_3D ( 'NONE', #114102, #24434, #103645 ) ;
#79813=DIRECTION ( 'NONE',  ( -0.000000000000000000, 1.000000000000000000, -0.000000000000000000 ) ) ;
#79814=CARTESIAN_POINT ( 'NONE',  ( 8.299999999999922551, 2.500000000000000000, 4.330127018922196314 ) ) ;
#79815=EDGE_CURVE ( 'NONE', #57530, #95831, #105255, .T. ) ;
#79816=AXIS2_PLACEMENT_3D ( 'NONE', #92743, #3074, #54100 ) ;
#79817=VERTEX_POINT ( 'NONE', #76992 ) ;
#79818=CARTESIAN_POINT ( 'NONE',  ( -2.050000000000033129, 2.500000000000000000, 6.495190528383297135 ) ) ;
#79819=EDGE_LOOP ( 'NONE', ( #53555, #45838 ) ) ;
#79820=ORIENTED_EDGE ( 'NONE', *, *, #75105, .F. ) ;
#79821=CARTESIAN_POINT ( 'NONE',  ( -11.05000000000000071, 12.50000000000000000, 6.841600689897072485 ) ) ;
#79822=ADVANCED_FACE ( 'NONE', ( #17404 ), #58010, .T. ) ;
#79823=DIRECTION ( 'NONE',  ( -0.000000000000000000, -1.000000000000000000, -0.000000000000000000 ) ) ;
#79824=FACE_BOUND ( 'NONE', #30730, .T. ) ;
#79825=DIRECTION ( 'NONE',  ( 0.000000000000000000, 0.000000000000000000, 1.000000000000000000 ) ) ;
#79826=DIRECTION ( 'NONE',  ( -0.000000000000000000, 1.000000000000000000, -0.000000000000000000 ) ) ;
#79827=LINE ( 'NONE', #82431, #79279 ) ;
#79828=LINE ( 'NONE', #2541, #71374 ) ;
#79829=DIRECTION ( 'NONE',  ( 0.000000000000000000, -0.000000000000000000, 1.000000000000000000 ) ) ;
#79832=ORIENTED_EDGE ( 'NONE', *, *, #33479, .F. ) ;
#79833=VECTOR ( 'NONE', #43596, 1000.000000000000000 ) ;
#79834=LINE ( 'NONE', #66782, #19782 ) ;
#79835=CIRCLE ( 'NONE', #71414, 0.06509327318403745899 ) ;
#79836=LINE ( 'NONE', #91596, #129058 ) ;
#79837=ORIENTED_EDGE ( 'NONE', *, *, #27842, .T. ) ;
#79838=ORIENTED_EDGE ( 'NONE', *, *, #64388, .F. ) ;
#79840=CARTESIAN_POINT ( 'NONE',  ( -5.200000000000024158, 12.50000000000000000, -4.741630453620015118 ) ) ;
#79841=FACE_BOUND ( 'NONE', #48530, .T. ) ;
#79842=VECTOR ( 'NONE', #121496, 1000.000000000000000 ) ;
#79843=DIRECTION ( 'NONE',  ( 0.000000000000000000, 0.000000000000000000, 1.000000000000000000 ) ) ;
#79844=AXIS2_PLACEMENT_3D ( 'NONE', #34889, #124542, #57068 ) ;
#79845=EDGE_CURVE ( 'NONE', #71852, #68242, #97913, .T. ) ;
#79846=CIRCLE ( 'NONE', #77776, 0.06509327318403745899 ) ;
#79847=DIRECTION ( 'NONE',  ( -0.000000000000000000, 1.000000000000000000, -0.000000000000000000 ) ) ;
#79848=ORIENTED_EDGE ( 'NONE', *, *, #24614, .T. ) ;
#79849=CARTESIAN_POINT ( 'NONE',  ( 10.19999999999991580, 2.500000000000000000, -0.2464101615137783419 ) ) ;
#79850=EDGE_CURVE ( 'NONE', #15541, #66128, #73865, .T. ) ;
#79851=DIRECTION ( 'NONE',  ( 0.000000000000000000, 0.000000000000000000, 1.000000000000000000 ) ) ;
#79852=EDGE_CURVE ( 'NONE', #14663, #59275, #57352, .T. ) ;
#79853=ORIENTED_EDGE ( 'NONE', *, *, #18056, .T. ) ;
#79854=VECTOR ( 'NONE', #125062, 1000.000000000000000 ) ;
#79855=LINE ( 'NONE', #108023, #103267 ) ;
#79856=DIRECTION ( 'NONE',  ( -4.274815082592931898E-19, -0.9999939076577903929, -0.003490651415223739937 ) ) ;
#79857=CIRCLE ( 'NONE', #17126, 0.06509327318403745899 ) ;
#79858=CIRCLE ( 'NONE', #17129, 0.06509327318403745899 ) ;
#79860=AXIS2_PLACEMENT_3D ( 'NONE', #62980, #93100, #11940 ) ;
#79861=ADVANCED_FACE ( 'NONE', ( #59310 ), #67140, .T. ) ;
#79862=EDGE_CURVE ( 'NONE', #85603, #96773, #34169, .T. ) ;
#79863=CARTESIAN_POINT ( 'NONE',  ( 10.39999999999990976, 12.50000000000000000, -4.265033745738164406 ) ) ;
#79864=EDGE_CURVE ( 'NONE', #73360, #57691, #17410, .T. ) ;
#79865=CARTESIAN_POINT ( 'NONE',  ( 9.599999999999914380, 2.500000000000000000, 3.737306695894644371 ) ) ;
#79866=AXIS2_PLACEMENT_3D ( 'NONE', #37358, #18342, #126372 ) ;
#79867=ORIENTED_EDGE ( 'NONE', *, *, #55614, .T. ) ;
#79868=DIRECTION ( 'NONE',  ( 0.000000000000000000, 0.000000000000000000, 1.000000000000000000 ) ) ;
#79869=ADVANCED_FACE ( 'NONE', ( #128027 ), #61356, .T. ) ;
#79870=AXIS2_PLACEMENT_3D ( 'NONE', #76646, #26262, #126392 ) ;
#79871=CARTESIAN_POINT ( 'NONE',  ( 8.149999999999920419, 2.500000000000000000, -2.411473670974877859 ) ) ;
#79872=CARTESIAN_POINT ( 'NONE',  ( -5.450000000000019718, 12.50000000000000000, 6.495190528383297135 ) ) ;
#79873=CARTESIAN_POINT ( 'NONE',  ( 6.649999999999931966, 2.500000000000000000, -7.188010851410854052 ) ) ;
#79875=EDGE_LOOP ( 'NONE', ( #102256, #112794 ) ) ;
#79876=CARTESIAN_POINT ( 'NONE',  ( 1.899999999999951283, 12.50000000000000000, -4.676537180435977881 ) ) ;
#79877=EDGE_CURVE ( 'NONE', #1361, #112572, #11163, .T. ) ;
#79878=ORIENTED_EDGE ( 'NONE', *, *, #37157, .T. ) ;
#79879=CARTESIAN_POINT ( 'NONE',  ( -3.300000000000027800, 12.50000000000000000, -2.276824562219559311E-15 ) ) ;
#79880=CARTESIAN_POINT ( 'NONE',  ( 17.50000000000000000, -2.499999999999999556, 0.3333333333333385884 ) ) ;
#79881=FACE_OUTER_BOUND ( 'NONE', #75958, .T. ) ;
#79884=DIRECTION ( 'NONE',  ( 0.000000000000000000, 0.000000000000000000, 1.000000000000000000 ) ) ;
#79885=FACE_OUTER_BOUND ( 'NONE', #64101, .T. ) ;
#79886=DIRECTION ( 'NONE',  ( -0.000000000000000000, 1.000000000000000000, -0.000000000000000000 ) ) ;
#79887=CARTESIAN_POINT ( 'NONE',  ( 13.54999999999989946, 12.50000000000000000, 2.446380397790835826 ) ) ;
#79888=CARTESIAN_POINT ( 'NONE',  ( -10.85000000000000142, 2.500000000000000000, 2.065063509461097624 ) ) ;
#79889=ORIENTED_EDGE ( 'NONE', *, *, #4841, .F. ) ;
#79890=ORIENTED_EDGE ( 'NONE', *, *, #114616, .T. ) ;
#79891=DIRECTION ( 'NONE',  ( 0.000000000000000000, 0.000000000000000000, -1.000000000000000000 ) ) ;
#79892=ORIENTED_EDGE ( 'NONE', *, *, #49495, .F. ) ;
#79893=AXIS2_PLACEMENT_3D ( 'NONE', #50235, #9652, #49596 ) ;
#79894=CARTESIAN_POINT ( 'NONE',  ( 12.89999999999989910, 2.500000000000000000, -0.6928203230275542523 ) ) ;
#79895=AXIS2_PLACEMENT_3D ( 'NONE', #126508, #85284, #66291 ) ;
#79896=CIRCLE ( 'NONE', #31788, 0.06509327318403745899 ) ;
#79897=ORIENTED_EDGE ( 'NONE', *, *, #81459, .F. ) ;
#79898=EDGE_LOOP ( 'NONE', ( #103568, #10862 ) ) ;
#79899=VERTEX_POINT ( 'NONE', #78301 ) ;
#79900=CARTESIAN_POINT ( 'NONE',  ( 17.50000000000000000, 0.4166666666666715146, -3.999999999999996447 ) ) ;
#79901=DIRECTION ( 'NONE',  ( -4.274815082592931898E-19, -0.9999939076577903929, -0.003490651415223739937 ) ) ;
#79902=AXIS2_PLACEMENT_3D ( 'NONE', #129438, #107832, #99308 ) ;
#79903=VECTOR ( 'NONE', #63534, 1000.000000000000000 ) ;
#79904=DIRECTION ( 'NONE',  ( 0.000000000000000000, 0.000000000000000000, 1.000000000000000000 ) ) ;
#79905=CONICAL_SURFACE ( 'NONE', #67347, 0.09999999999999982514, 0.003490658503988666988 ) ;
#79906=DIRECTION ( 'NONE',  ( 0.000000000000000000, 0.000000000000000000, 1.000000000000000000 ) ) ;
#79907=DIRECTION ( 'NONE',  ( 0.000000000000000000, -0.000000000000000000, 1.000000000000000000 ) ) ;
#79908=DIRECTION ( 'NONE',  ( -0.000000000000000000, -1.000000000000000000, -0.000000000000000000 ) ) ;
#79909=AXIS2_PLACEMENT_3D ( 'NONE', #48031, #128540, #9384 ) ;
#79910=FACE_OUTER_BOUND ( 'NONE', #53659, .T. ) ;
#79911=FACE_OUTER_BOUND ( 'NONE', #71874, .T. ) ;
#79912=CONICAL_SURFACE ( 'NONE', #84101, 0.09999999999999982514, 0.003490658503988666988 ) ;
#79913=CARTESIAN_POINT ( 'NONE',  ( 9.149999999999915090, 2.500000000000000000, 6.395190528383296602 ) ) ;
#79914=CIRCLE ( 'NONE', #12989, 0.06509327318403743123 ) ;
#79915=ORIENTED_EDGE ( 'NONE', *, *, #66583, .T. ) ;
#79916=VERTEX_POINT ( 'NONE', #51424 ) ;
#79917=ADVANCED_FACE ( 'NONE', ( #110321 ), #91970, .T. ) ;
#79918=DIRECTION ( 'NONE',  ( 0.000000000000000000, 0.000000000000000000, 1.000000000000000000 ) ) ;
#79919=VERTEX_POINT ( 'NONE', #91323 ) ;
#79920=VERTEX_POINT ( 'NONE', #20660 ) ;
#79921=CARTESIAN_POINT ( 'NONE',  ( 4.599999999999936584, 2.500000000000000000, 3.537306695894645081 ) ) ;
#79922=ADVANCED_FACE ( 'NONE', ( #22608 ), #84330, .T. ) ;
#79924=DIRECTION ( 'NONE',  ( 0.000000000000000000, 0.000000000000000000, 1.000000000000000000 ) ) ;
#79925=CARTESIAN_POINT ( 'NONE',  ( -13.14999999999999147, 2.500000000000000000, -1.918653347947324006 ) ) ;
#79926=CARTESIAN_POINT ( 'NONE',  ( 12.49999999999993960, 12.50000000000000000, -4.330127018922201643 ) ) ;
#79927=ORIENTED_EDGE ( 'NONE', *, *, #29583, .T. ) ;
#79928=AXIS2_PLACEMENT_3D ( 'NONE', #107659, #67051, #48093 ) ;
#79929=VERTEX_POINT ( 'NONE', #21963 ) ;
#79930=DIRECTION ( 'NONE',  ( 0.000000000000000000, 0.000000000000000000, 1.000000000000000000 ) ) ;
#79931=ORIENTED_EDGE ( 'NONE', *, *, #9519, .F. ) ;
#79932=CARTESIAN_POINT ( 'NONE',  ( 13.54999999999989591, 12.50000000000000000, -1.818653347947326138 ) ) ;
#79933=ORIENTED_EDGE ( 'NONE', *, *, #109678, .T. ) ;
#79934=ORIENTED_EDGE ( 'NONE', *, *, #100125, .T. ) ;
#79935=CIRCLE ( 'NONE', #17207, 0.09999999999999999167 ) ;
#79936=CARTESIAN_POINT ( 'NONE',  ( 11.84999999999990727, 12.50000000000000000, 6.083687093685482772 ) ) ;
#79937=CARTESIAN_POINT ( 'NONE',  ( 3.149999999999946176, 2.500000000000000000, -2.611473670974877592 ) ) ;
#79938=AXIS2_PLACEMENT_3D ( 'NONE', #31009, #70910, #101003 ) ;
#79939=CARTESIAN_POINT ( 'NONE',  ( -6.650000000000014566, 12.50000000000000000, 6.495190528383297135 ) ) ;
#79940=CIRCLE ( 'NONE', #21449, 0.1000000000000002554 ) ;
#79941=CARTESIAN_POINT ( 'NONE',  ( -1.250000000000001554, 2.500000000000000000, 6.495190528383297135 ) ) ;
#79942=CARTESIAN_POINT ( 'NONE',  ( 17.50000000000000000, -0.4166666666666683505, 4.000000000000001776 ) ) ;
#79943=EDGE_LOOP ( 'NONE', ( #37791, #29843 ) ) ;
#79944=CARTESIAN_POINT ( 'NONE',  ( -1.700000000000035261, 12.50000000000000000, 4.330127018922196314 ) ) ;
#79945=CARTESIAN_POINT ( 'NONE',  ( -7.900000000000011013, 2.500000000000000000, 5.122947341949749323 ) ) ;
#79946=DIRECTION ( 'NONE',  ( -4.274815082592931898E-19, -0.9999939076577903929, -0.003490651415223739937 ) ) ;
#79947=DIRECTION ( 'NONE',  ( 0.000000000000000000, 0.000000000000000000, 1.000000000000000000 ) ) ;
#79948=VECTOR ( 'NONE', #111204, 1000.000000000000000 ) ;
#79949=AXIS2_PLACEMENT_3D ( 'NONE', #70189, #110743, #10593 ) ;
#79950=CARTESIAN_POINT ( 'NONE',  ( -12.89999999999999147, 2.500000000000000000, -0.6928203230275500335 ) ) ;
#79951=ADVANCED_FACE ( 'NONE', ( #31139 ), #69755, .T. ) ;
#79952=ORIENTED_EDGE ( 'NONE', *, *, #35621, .T. ) ;
#79953=AXIS2_PLACEMENT_3D ( 'NONE', #108570, #80412, #60764 ) ;
#79954=AXIS2_PLACEMENT_3D ( 'NONE', #12453, #1349, #52388 ) ;
#79955=VECTOR ( 'NONE', #28869, 1000.000000000000000 ) ;
#79956=VERTEX_POINT ( 'NONE', #71044 ) ;
#79957=LINE ( 'NONE', #12500, #54945 ) ;
#79958=CIRCLE ( 'NONE', #23516, 0.06509327318403745899 ) ;
#79959=VERTEX_POINT ( 'NONE', #109683 ) ;
#79960=DIRECTION ( 'NONE',  ( -0.000000000000000000, 1.000000000000000000, -0.000000000000000000 ) ) ;
#79961=DIRECTION ( 'NONE',  ( -0.000000000000000000, 1.000000000000000000, -0.000000000000000000 ) ) ;
#79962=EDGE_CURVE ( 'NONE', #65030, #102327, #101057, .T. ) ;
#79963=AXIS2_PLACEMENT_3D ( 'NONE', #60249, #72632, #62810 ) ;
#79964=ADVANCED_FACE ( 'NONE', ( #71683 ), #55183, .T. ) ;
#79965=ORIENTED_EDGE ( 'NONE', *, *, #77345, .T. ) ;
#79966=DIRECTION ( 'NONE',  ( 0.000000000000000000, 0.000000000000000000, 1.000000000000000000 ) ) ;
#79967=CARTESIAN_POINT ( 'NONE',  ( 15.19999999999989093, 2.500000000000000000, 0.3464101615137735735 ) ) ;
#79968=EDGE_CURVE ( 'NONE', #224, #91651, #53040, .T. ) ;
#79969=CARTESIAN_POINT ( 'NONE',  ( -3.950000000000029932, 12.50000000000000000, -6.148780366869526226 ) ) ;
#79970=CARTESIAN_POINT ( 'NONE',  ( -10.80000000000000249, 12.50000000000000000, -4.395220292106235327 ) ) ;
#79971=EDGE_CURVE ( 'NONE', #125180, #66966, #2283, .T. ) ;
#79972=EDGE_LOOP ( 'NONE', ( #41772, #73219, #35622, #107973 ) ) ;
#79973=VECTOR ( 'NONE', #102168, 1000.000000000000000 ) ;
#79974=EDGE_CURVE ( 'NONE', #101819, #102850, #110944, .T. ) ;
#79975=CARTESIAN_POINT ( 'NONE',  ( 23.85228139349051091, 2.660541499546454247, -4.258215071919995154 ) ) ;
#79976=FACE_OUTER_BOUND ( 'NONE', #14304, .T. ) ;
#79977=FACE_OUTER_BOUND ( 'NONE', #69529, .T. ) ;
#79978=VERTEX_POINT ( 'NONE', #82154 ) ;
#79979=DIRECTION ( 'NONE',  ( 0.000000000000000000, 0.000000000000000000, 1.000000000000000000 ) ) ;
#79980=VECTOR ( 'NONE', #19303, 1000.000000000000000 ) ;
#79982=AXIS2_PLACEMENT_3D ( 'NONE', #42272, #101830, #122121 ) ;
#79983=VERTEX_POINT ( 'NONE', #101151 ) ;
#79984=CARTESIAN_POINT ( 'NONE',  ( 10.79999999999991367, 2.500000000000000000, -0.1000000000000023925 ) ) ;
#79985=DIRECTION ( 'NONE',  ( 0.000000000000000000, 1.000000000000000000, 0.000000000000000000 ) ) ;
#79986=LINE ( 'NONE', #120561, #81020 ) ;
#79987=VERTEX_POINT ( 'NONE', #62527 ) ;
#79988=VECTOR ( 'NONE', #72688, 1000.000000000000000 ) ;
#79989=LINE ( 'NONE', #27646, #40548 ) ;
#79991=VECTOR ( 'NONE', #125975, 1000.000000000000000 ) ;
#79992=DIRECTION ( 'NONE',  ( -4.274815082592931898E-19, -0.9999939076577903929, -0.003490651415223739937 ) ) ;
#79993=CIRCLE ( 'NONE', #8878, 0.06509327318403745899 ) ;
#79994=VERTEX_POINT ( 'NONE', #119484 ) ;
#79995=CIRCLE ( 'NONE', #31991, 0.06509327318403745899 ) ;
#79996=DIRECTION ( 'NONE',  ( 0.000000000000000000, 1.000000000000000000, 0.000000000000000000 ) ) ;
#79997=ORIENTED_EDGE ( 'NONE', *, *, #24033, .T. ) ;
#79998=CIRCLE ( 'NONE', #125965, 0.06509327318403745899 ) ;
#79999=CARTESIAN_POINT ( 'NONE',  ( -10.20000000000000284, 2.500000000000000000, -0.4464101615137782142 ) ) ;
#80000=EDGE_CURVE ( 'NONE', #29710, #55568, #21733, .T. ) ;
#80002=DIRECTION ( 'NONE',  ( -0.000000000000000000, 1.000000000000000000, -0.000000000000000000 ) ) ;
#80003=DIRECTION ( 'NONE',  ( -0.000000000000000000, -1.000000000000000000, -0.000000000000000000 ) ) ;
#80004=EDGE_LOOP ( 'NONE', ( #63458, #25864 ) ) ;
#80005=ORIENTED_EDGE ( 'NONE', *, *, #71246, .F. ) ;
#80006=DIRECTION ( 'NONE',  ( 0.000000000000000000, 1.000000000000000000, 0.000000000000000000 ) ) ;
#80007=DIRECTION ( 'NONE',  ( -0.000000000000000000, 1.000000000000000000, -0.000000000000000000 ) ) ;
#80008=ORIENTED_EDGE ( 'NONE', *, *, #29625, .F. ) ;
#80009=ADVANCED_FACE ( 'NONE', ( #122084 ), #29831, .T. ) ;
#80010=CIRCLE ( 'NONE', #71698, 0.09999999999999999167 ) ;
#80011=DIRECTION ( 'NONE',  ( 0.000000000000000000, 0.000000000000000000, 1.000000000000000000 ) ) ;
#80012=FACE_OUTER_BOUND ( 'NONE', #84450, .T. ) ;
#80013=CARTESIAN_POINT ( 'NONE',  ( -4.150000000000025224, 2.500000000000000000, 6.495190528383297135 ) ) ;
#80014=DIRECTION ( 'NONE',  ( 0.000000000000000000, 0.000000000000000000, 1.000000000000000000 ) ) ;
#80015=PLANE ( 'NONE',  #15342 ) ;
#80016=EDGE_CURVE ( 'NONE', #123447, #69623, #39675, .T. ) ;
#80017=DIRECTION ( 'NONE',  ( 0.000000000000000000, -0.9999939076577903929, 0.003490651415223739937 ) ) ;
#80018=FACE_OUTER_BOUND ( 'NONE', #14845, .T. ) ;
#80019=EDGE_CURVE ( 'NONE', #103166, #122201, #52689, .T. ) ;
#80020=EDGE_CURVE ( 'NONE', #119523, #23602, #34270, .T. ) ;
#80021=AXIS2_PLACEMENT_3D ( 'NONE', #75446, #115353, #25709 ) ;
#80022=AXIS2_PLACEMENT_3D ( 'NONE', #10148, #89981, #78259 ) ;
#80023=VERTEX_POINT ( 'NONE', #59964 ) ;
#80024=ORIENTED_EDGE ( 'NONE', *, *, #84833, .F. ) ;
#80025=EDGE_CURVE ( 'NONE', #26527, #3072, #126188, .T. ) ;
#80026=ORIENTED_EDGE ( 'NONE', *, *, #93004, .F. ) ;
#80027=CARTESIAN_POINT ( 'NONE',  ( 7.049999999999930544, 12.50000000000000000, -6.560283801567339701 ) ) ;
#80028=FACE_OUTER_BOUND ( 'NONE', #63953, .T. ) ;
#80029=DIRECTION ( 'NONE',  ( 0.000000000000000000, 0.000000000000000000, -1.000000000000000000 ) ) ;
#80030=ORIENTED_EDGE ( 'NONE', *, *, #2270, .F. ) ;
#80031=FACE_BOUND ( 'NONE', #23189, .T. ) ;
#80032=EDGE_LOOP ( 'NONE', ( #1736, #1665 ) ) ;
#80033=AXIS2_PLACEMENT_3D ( 'NONE', #38650, #119757, #80500 ) ;
#80034=DIRECTION ( 'NONE',  ( 0.000000000000000000, -0.000000000000000000, 1.000000000000000000 ) ) ;
#80035=DIRECTION ( 'NONE',  ( 0.000000000000000000, 0.000000000000000000, -1.000000000000000000 ) ) ;
#80036=ADVANCED_FACE ( 'NONE', ( #10191 ), #17507, .T. ) ;
#80037=LINE ( 'NONE', #120606, #30491 ) ;
#80038=EDGE_CURVE ( 'NONE', #50530, #124116, #33072, .T. ) ;
#80039=CONICAL_SURFACE ( 'NONE', #25740, 0.1000000000000002554, 0.003490658503988666988 ) ;
#80040=DIRECTION ( 'NONE',  ( 0.000000000000000000, 0.000000000000000000, -1.000000000000000000 ) ) ;
#80041=DIRECTION ( 'NONE',  ( -4.274815082592931898E-19, -0.9999939076577903929, -0.003490651415223739937 ) ) ;
#80042=DIRECTION ( 'NONE',  ( -4.274815082592931898E-19, -0.9999939076577903929, -0.003490651415223739937 ) ) ;
#80043=CARTESIAN_POINT ( 'NONE',  ( 11.89999999999990798, 12.50000000000000000, 3.983716857408420964 ) ) ;
#80044=LINE ( 'NONE', #87905, #53651 ) ;
#80045=VECTOR ( 'NONE', #103988, 1000.000000000000000 ) ;
#80046=CARTESIAN_POINT ( 'NONE',  ( 8.299999999999922551, 2.500000000000000000, -4.330127018922201643 ) ) ;
#80047=AXIS2_PLACEMENT_3D ( 'NONE', #6559, #107378, #46510 ) ;
#80048=ORIENTED_EDGE ( 'NONE', *, *, #90174, .F. ) ;
#80049=ORIENTED_EDGE ( 'NONE', *, *, #53627, .F. ) ;
#80050=VERTEX_POINT ( 'NONE', #75534 ) ;
#80051=AXIS2_PLACEMENT_3D ( 'NONE', #62706, #61426, #52237 ) ;
#80052=ORIENTED_EDGE ( 'NONE', *, *, #70151, .F. ) ;
#80053=CIRCLE ( 'NONE', #123949, 0.1000000000000002554 ) ;
#80054=CONICAL_SURFACE ( 'NONE', #117583, 0.09999999999999982514, 0.003490658503988666988 ) ;
#80055=CARTESIAN_POINT ( 'NONE',  ( -4.150000000000025224, 2.500000000000000000, 5.802370205355744659 ) ) ;
#80056=LINE ( 'NONE', #2779, #13078 ) ;
#80057=ORIENTED_EDGE ( 'NONE', *, *, #24851, .T. ) ;
#80058=ORIENTED_EDGE ( 'NONE', *, *, #66152, .F. ) ;
#80061=CARTESIAN_POINT ( 'NONE',  ( -4.999999999999986677, 2.500000000000000000, -0.1000000000000022815 ) ) ;
#80062=DIRECTION ( 'NONE',  ( 0.000000000000000000, 0.000000000000000000, 1.000000000000000000 ) ) ;
#80063=VECTOR ( 'NONE', #129488, 1000.000000000000000 ) ;
#80064=CARTESIAN_POINT ( 'NONE',  ( 5.599999999999933031, 2.500000000000000000, 0.3464101615137735735 ) ) ;
#80065=DIRECTION ( 'NONE',  ( 0.000000000000000000, 0.000000000000000000, 1.000000000000000000 ) ) ;
#80068=LINE ( 'NONE', #9399, #46846 ) ;
#80069=EDGE_LOOP ( 'NONE', ( #37073, #106041, #71327, #75926 ) ) ;
#80070=DIRECTION ( 'NONE',  ( 0.000000000000000000, -0.000000000000000000, 1.000000000000000000 ) ) ;
#80071=ORIENTED_EDGE ( 'NONE', *, *, #69957, .F. ) ;
#80072=EDGE_LOOP ( 'NONE', ( #87592, #77591, #83923, #9104 ) ) ;
#80073=ADVANCED_FACE ( 'NONE', ( #124661 ), #63151, .T. ) ;
#80074=ORIENTED_EDGE ( 'NONE', *, *, #25808, .F. ) ;
#80075=CARTESIAN_POINT ( 'NONE',  ( -3.950000000000026379, 2.500000000000000000, 6.841600689897072485 ) ) ;
#80076=AXIS2_PLACEMENT_3D ( 'NONE', #54615, #64443, #114824 ) ;
#80077=VECTOR ( 'NONE', #66741, 1000.000000000000000 ) ;
#80078=EDGE_LOOP ( 'NONE', ( #42168, #6969, #29144, #21118, #48149 ) ) ;
#80079=VERTEX_POINT ( 'NONE', #2952 ) ;
#80080=DIRECTION ( 'NONE',  ( 0.000000000000000000, 0.000000000000000000, -1.000000000000000000 ) ) ;
#80081=ADVANCED_FACE ( 'NONE', ( #14676 ), #117852, .T. ) ;
#80082=CIRCLE ( 'NONE', #86609, 0.06509327318403745899 ) ;
#80083=CARTESIAN_POINT ( 'NONE',  ( 2.049999999999948308, 2.500000000000000000, 6.395190528383296602 ) ) ;
#80084=DIRECTION ( 'NONE',  ( -0.000000000000000000, -1.000000000000000000, -0.000000000000000000 ) ) ;
#80085=CIRCLE ( 'NONE', #103059, 0.06509327318403745899 ) ;
#80086=DIRECTION ( 'NONE',  ( 0.000000000000000000, 1.000000000000000000, 0.000000000000000000 ) ) ;
#80087=VECTOR ( 'NONE', #128196, 1000.000000000000000 ) ;
#80088=CIRCLE ( 'NONE', #88370, 0.06509327318403741736 ) ;
#80089=DIRECTION ( 'NONE',  ( 0.000000000000000000, 1.000000000000000000, 0.000000000000000000 ) ) ;
#80090=VERTEX_POINT ( 'NONE', #115449 ) ;
#80091=CARTESIAN_POINT ( 'NONE',  ( -5.650000000000019895, 12.50000000000000000, 2.511473670974873507 ) ) ;
#80092=AXIS2_PLACEMENT_3D ( 'NONE', #88273, #46431, #128244 ) ;
#80093=CIRCLE ( 'NONE', #40393, 0.1000000000000000472 ) ;
#80094=ORIENTED_EDGE ( 'NONE', *, *, #40736, .F. ) ;
#80095=FACE_OUTER_BOUND ( 'NONE', #1839, .T. ) ;
#80096=CIRCLE ( 'NONE', #4857, 0.06509327318403745899 ) ;
#80097=ORIENTED_EDGE ( 'NONE', *, *, #41947, .T. ) ;
#80098=DIRECTION ( 'NONE',  ( 0.000000000000000000, 0.000000000000000000, -1.000000000000000000 ) ) ;
#80099=DIRECTION ( 'NONE',  ( -4.274815082592931898E-19, -0.9999939076577903929, -0.003490651415223739937 ) ) ;
#80100=CIRCLE ( 'NONE', #103077, 0.06509327318403745899 ) ;
#80101=ORIENTED_EDGE ( 'NONE', *, *, #18016, .F. ) ;
#80102=AXIS2_PLACEMENT_3D ( 'NONE', #38747, #97634, #77994 ) ;
#80103=CARTESIAN_POINT ( 'NONE',  ( 3.099999999999945466, 12.50000000000000000, 0.3464101615137735735 ) ) ;
#80104=LINE ( 'NONE', #8756, #125174 ) ;
#80106=AXIS2_PLACEMENT_3D ( 'NONE', #37459, #117926, #46612 ) ;
#80107=CARTESIAN_POINT ( 'NONE',  ( -7.100000000000017408, 2.500000000000000000, 0.7928203230275495672 ) ) ;
#80108=ORIENTED_EDGE ( 'NONE', *, *, #69046, .T. ) ;
#80109=ORIENTED_EDGE ( 'NONE', *, *, #13520, .F. ) ;
#80110=DIRECTION ( 'NONE',  ( 0.000000000000000000, -0.9999939076577903929, 0.003490651415223739937 ) ) ;
#80111=DIRECTION ( 'NONE',  ( 0.000000000000000000, -0.9999939076577903929, 0.003490651415223739937 ) ) ;
#80113=DIRECTION ( 'NONE',  ( -0.000000000000000000, -1.000000000000000000, -0.000000000000000000 ) ) ;
#80114=CONICAL_SURFACE ( 'NONE', #69643, 0.09999999999999982514, 0.003490658503988666988 ) ;
#80115=DIRECTION ( 'NONE',  ( 0.000000000000000000, 0.000000000000000000, -1.000000000000000000 ) ) ;
#80116=VERTEX_POINT ( 'NONE', #85369 ) ;
#80118=ORIENTED_EDGE ( 'NONE', *, *, #129442, .F. ) ;
#80119=AXIS2_PLACEMENT_3D ( 'NONE', #112862, #61182, #2911 ) ;
#80120=DIRECTION ( 'NONE',  ( 0.000000000000000000, 0.000000000000000000, 1.000000000000000000 ) ) ;
#80121=DIRECTION ( 'NONE',  ( 0.000000000000000000, 0.000000000000000000, 1.000000000000000000 ) ) ;
#80122=EDGE_CURVE ( 'NONE', #17444, #43807, #74267, .T. ) ;
#80123=CIRCLE ( 'NONE', #96830, 0.06509327318403745899 ) ;
#80124=EDGE_CURVE ( 'NONE', #117313, #38438, #25807, .T. ) ;
#80125=DIRECTION ( 'NONE',  ( 0.000000000000000000, 0.000000000000000000, 1.000000000000000000 ) ) ;
#80127=CARTESIAN_POINT ( 'NONE',  ( -8.100000000000013856, 2.500000000000000000, 0.3464101615137736845 ) ) ;
#80128=DIRECTION ( 'NONE',  ( -0.000000000000000000, -1.000000000000000000, -0.000000000000000000 ) ) ;
#80129=CIRCLE ( 'NONE', #73863, 0.06509327318403745899 ) ;
#80130=EDGE_CURVE ( 'NONE', #66886, #107927, #44815, .T. ) ;
#80131=LINE ( 'NONE', #260, #49615 ) ;
#80132=CIRCLE ( 'NONE', #82285, 0.06509327318403745899 ) ;
#80133=VERTEX_POINT ( 'NONE', #84722 ) ;
#80134=VECTOR ( 'NONE', #51722, 1000.000000000000000 ) ;
#80135=CIRCLE ( 'NONE', #13214, 0.06509327318403745899 ) ;
#80136=DIRECTION ( 'NONE',  ( 0.000000000000000000, 0.000000000000000000, -1.000000000000000000 ) ) ;
#80137=CARTESIAN_POINT ( 'NONE',  ( 13.94999999999989448, 2.500000000000000000, -2.411473670974877859 ) ) ;
#80138=CARTESIAN_POINT ( 'NONE',  ( 13.54999999999989768, 12.50000000000000000, -2.511473670974877948 ) ) ;
#80139=EDGE_CURVE ( 'NONE', #32427, #91045, #30059, .T. ) ;
#80140=EDGE_CURVE ( 'NONE', #32930, #92950, #82385, .T. ) ;
#80141=EDGE_CURVE ( 'NONE', #45961, #11906, #122089, .T. ) ;
#80142=ORIENTED_EDGE ( 'NONE', *, *, #31755, .T. ) ;
#80143=CARTESIAN_POINT ( 'NONE',  ( -4.350000000000023626, 2.500000000000000000, 6.248780366869521430 ) ) ;
#80144=EDGE_LOOP ( 'NONE', ( #14400, #6159 ) ) ;
#80145=CIRCLE ( 'NONE', #84345, 0.06509327318403745899 ) ;
#80146=VERTEX_POINT ( 'NONE', #72976 ) ;
#80147=CIRCLE ( 'NONE', #121912, 0.06509327318403745899 ) ;
#80148=DIRECTION ( 'NONE',  ( -0.000000000000000000, -1.000000000000000000, -0.000000000000000000 ) ) ;
#80149=VECTOR ( 'NONE', #107713, 1000.000000000000000 ) ;
#80150=ORIENTED_EDGE ( 'NONE', *, *, #9910, .T. ) ;
#80151=CARTESIAN_POINT ( 'NONE',  ( -7.100000000000018296, 2.500000000000000000, -0.1000000000000023925 ) ) ;
#80152=CARTESIAN_POINT ( 'NONE',  ( -3.100000000000028511, 12.50000000000000000, 0.3464101615137736845 ) ) ;
#80153=ORIENTED_EDGE ( 'NONE', *, *, #23426, .T. ) ;
#80154=DIRECTION ( 'NONE',  ( 0.000000000000000000, -0.9999939076577903929, 0.003490651415223739937 ) ) ;
#80155=CARTESIAN_POINT ( 'NONE',  ( -9.150000000000009237, 2.500000000000000000, 2.857883832488649301 ) ) ;
#80156=ORIENTED_EDGE ( 'NONE', *, *, #114205, .F. ) ;
#80158=ORIENTED_EDGE ( 'NONE', *, *, #61293, .T. ) ;
#80159=DIRECTION ( 'NONE',  ( 0.000000000000000000, 0.000000000000000000, 1.000000000000000000 ) ) ;
#80160=CARTESIAN_POINT ( 'NONE',  ( 6.699999999999930012, 2.500000000000000000, 4.330127018922196314 ) ) ;
#80161=AXIS2_PLACEMENT_3D ( 'NONE', #105353, #47090, #37895 ) ;
#80162=PLANE ( 'NONE',  #54718 ) ;
#80163=CIRCLE ( 'NONE', #67723, 0.06509327318403745899 ) ;
#80164=FACE_BOUND ( 'NONE', #61692, .T. ) ;
#80165=ORIENTED_EDGE ( 'NONE', *, *, #76594, .T. ) ;
#80166=DIRECTION ( 'NONE',  ( 0.000000000000000000, 0.000000000000000000, -1.000000000000000000 ) ) ;
#80167=DIRECTION ( 'NONE',  ( 0.000000000000000000, 0.000000000000000000, 1.000000000000000000 ) ) ;
#80168=ORIENTED_EDGE ( 'NONE', *, *, #37048, .F. ) ;
#80169=DIRECTION ( 'NONE',  ( 0.000000000000000000, 1.000000000000000000, 0.000000000000000000 ) ) ;
#80170=AXIS2_PLACEMENT_3D ( 'NONE', #12175, #61952, #92040 ) ;
#80171=DIRECTION ( 'NONE',  ( 0.000000000000000000, 1.000000000000000000, 0.000000000000000000 ) ) ;
#80172=AXIS2_PLACEMENT_3D ( 'NONE', #88451, #7962, #47910 ) ;
#80173=CONICAL_SURFACE ( 'NONE', #98955, 0.1000000000000000472, 0.003490658503988666988 ) ;
#80174=CARTESIAN_POINT ( 'NONE',  ( 14.99999999999989164, 2.500000000000000000, 0.7928203230275495672 ) ) ;
#80175=AXIS2_PLACEMENT_3D ( 'NONE', #38922, #98434, #59189 ) ;
#80176=EDGE_CURVE ( 'NONE', #56205, #83060, #4986, .T. ) ;
#80177=PLANE ( 'NONE',  #57151 ) ;
#80178=CARTESIAN_POINT ( 'NONE',  ( 1.649999999999949729, 2.500000000000000000, 5.802370205355744659 ) ) ;
#80179=ADVANCED_FACE ( 'NONE', ( #25152 ), #80230, .T. ) ;
#80180=FACE_OUTER_BOUND ( 'NONE', #69689, .T. ) ;
#80181=DIRECTION ( 'NONE',  ( -0.000000000000000000, 1.000000000000000000, -0.000000000000000000 ) ) ;
#80182=ADVANCED_FACE ( 'NONE', ( #33695 ), #38475, .T. ) ;
#80183=AXIS2_PLACEMENT_3D ( 'NONE', #14422, #74010, #66752 ) ;
#80184=AXIS2_PLACEMENT_3D ( 'NONE', #39522, #21133, #108227 ) ;
#80185=CIRCLE ( 'NONE', #11215, 0.06509327318403745899 ) ;
#80187=ORIENTED_EDGE ( 'NONE', *, *, #77544, .T. ) ;
#80188=EDGE_CURVE ( 'NONE', #120463, #84952, #23795, .T. ) ;
#80189=VERTEX_POINT ( 'NONE', #82811 ) ;
#80191=ORIENTED_EDGE ( 'NONE', *, *, #59026, .T. ) ;
#80192=CARTESIAN_POINT ( 'NONE',  ( -3.750000000000027978, 2.500000000000000000, 7.188010851410848723 ) ) ;
#80193=EDGE_CURVE ( 'NONE', #66198, #64623, #45466, .T. ) ;
#80194=CIRCLE ( 'NONE', #105318, 0.06509327318403745899 ) ;
#80195=FACE_OUTER_BOUND ( 'NONE', #40781, .T. ) ;
#80196=VERTEX_POINT ( 'NONE', #35636 ) ;
#80197=EDGE_CURVE ( 'NONE', #30016, #13274, #59407, .T. ) ;
#80198=FACE_BOUND ( 'NONE', #37997, .T. ) ;
#80199=DIRECTION ( 'NONE',  ( 0.000000000000000000, 0.000000000000000000, -1.000000000000000000 ) ) ;
#80200=EDGE_CURVE ( 'NONE', #97088, #76654, #23889, .T. ) ;
#80201=DIRECTION ( 'NONE',  ( 0.000000000000000000, 1.000000000000000000, 0.000000000000000000 ) ) ;
#80202=EDGE_CURVE ( 'NONE', #99291, #47871, #34357, .T. ) ;
#80203=FACE_OUTER_BOUND ( 'NONE', #6493, .T. ) ;
#80204=DIRECTION ( 'NONE',  ( 0.000000000000000000, 1.000000000000000000, 0.000000000000000000 ) ) ;
#80205=CARTESIAN_POINT ( 'NONE',  ( -9.999999999999969802, 2.500000000000000000, -2.276824562219559311E-15 ) ) ;
#80206=CARTESIAN_POINT ( 'NONE',  ( 0.3999999999999568345, 12.50000000000000000, -3.637306695894650055 ) ) ;
#80207=DIRECTION ( 'NONE',  ( 0.000000000000000000, 0.000000000000000000, 1.000000000000000000 ) ) ;
#80208=VERTEX_POINT ( 'NONE', #56543 ) ;
#80209=EDGE_CURVE ( 'NONE', #23974, #82534, #19675, .T. ) ;
#80210=AXIS2_PLACEMENT_3D ( 'NONE', #3361, #113310, #23645 ) ;
#80211=ORIENTED_EDGE ( 'NONE', *, *, #95102, .F. ) ;
#80212=ORIENTED_EDGE ( 'NONE', *, *, #63182, .F. ) ;
#80213=ORIENTED_EDGE ( 'NONE', *, *, #72482, .T. ) ;
#80214=VERTEX_POINT ( 'NONE', #48038 ) ;
#80215=EDGE_LOOP ( 'NONE', ( #48719, #100364 ) ) ;
#80216=DIRECTION ( 'NONE',  ( -4.274815082592931898E-19, -0.9999939076577903929, -0.003490651415223739937 ) ) ;
#80217=DIRECTION ( 'NONE',  ( 0.000000000000000000, 0.000000000000000000, 1.000000000000000000 ) ) ;
#80218=EDGE_LOOP ( 'NONE', ( #63843, #55390 ) ) ;
#80219=CARTESIAN_POINT ( 'NONE',  ( -8.350000000000013856, 2.500000000000000000, -2.165063509461101710 ) ) ;
#80220=CIRCLE ( 'NONE', #50673, 0.1000000000000000472 ) ;
#80221=CIRCLE ( 'NONE', #42578, 0.06509327318403745899 ) ;
#80222=CARTESIAN_POINT ( 'NONE',  ( -11.84999999999999787, 2.500000000000000000, -1.818653347947321919 ) ) ;
#80224=DIRECTION ( 'NONE',  ( -0.000000000000000000, -1.000000000000000000, -0.000000000000000000 ) ) ;
#80225=CARTESIAN_POINT ( 'NONE',  ( 1.449999999999952660, 12.50000000000000000, -6.841600689897078702 ) ) ;
#80226=CIRCLE ( 'NONE', #115810, 0.09999999999999982514 ) ;
#80227=VERTEX_POINT ( 'NONE', #76203 ) ;
#80228=DIRECTION ( 'NONE',  ( 0.000000000000000000, 0.000000000000000000, 1.000000000000000000 ) ) ;
#80229=CIRCLE ( 'NONE', #123832, 0.06509327318403745899 ) ;
#80230=CONICAL_SURFACE ( 'NONE', #115812, 0.09999999999999982514, 0.003490658503988666988 ) ;
#80231=VERTEX_POINT ( 'NONE', #6777 ) ;
#80232=VERTEX_POINT ( 'NONE', #16612 ) ;
#80233=LINE ( 'NONE', #48847, #78222 ) ;
#80234=DIRECTION ( 'NONE',  ( -0.000000000000000000, -1.000000000000000000, -0.000000000000000000 ) ) ;
#80235=DIRECTION ( 'NONE',  ( 0.000000000000000000, 0.000000000000000000, 1.000000000000000000 ) ) ;
#80236=VECTOR ( 'NONE', #97902, 1000.000000000000000 ) ;
#80237=EDGE_LOOP ( 'NONE', ( #49009, #128109, #17872, #95370 ) ) ;
#80238=ORIENTED_EDGE ( 'NONE', *, *, #117330, .F. ) ;
#80239=DIRECTION ( 'NONE',  ( -0.000000000000000000, 1.000000000000000000, -0.000000000000000000 ) ) ;
#80240=EDGE_CURVE ( 'NONE', #41669, #122705, #92846, .T. ) ;
#80242=AXIS2_PLACEMENT_3D ( 'NONE', #18490, #58435, #8649 ) ;
#80243=CARTESIAN_POINT ( 'NONE',  ( 7.949999999999922018, 2.500000000000000000, 6.595190528383296780 ) ) ;
#80244=AXIS2_PLACEMENT_3D ( 'NONE', #18993, #50398, #98851 ) ;
#80245=CONICAL_SURFACE ( 'NONE', #57253, 0.1000000000000002554, 0.003490658503988666988 ) ;
#80246=DIRECTION ( 'NONE',  ( -0.000000000000000000, -1.000000000000000000, -0.000000000000000000 ) ) ;
#80247=VERTEX_POINT ( 'NONE', #18564 ) ;
#80248=DIRECTION ( 'NONE',  ( 0.000000000000000000, 0.000000000000000000, 1.000000000000000000 ) ) ;
#80249=CIRCLE ( 'NONE', #51012, 0.06509327318403743123 ) ;
#80250=ORIENTED_EDGE ( 'NONE', *, *, #107484, .F. ) ;
#80251=CONICAL_SURFACE ( 'NONE', #7058, 0.1000000000000002554, 0.003490658503988666988 ) ;
#80252=DIRECTION ( 'NONE',  ( 0.000000000000000000, 1.000000000000000000, 0.000000000000000000 ) ) ;
#80253=EDGE_LOOP ( 'NONE', ( #82138, #32191, #4977, #106669 ) ) ;
#80255=CARTESIAN_POINT ( 'NONE',  ( -11.24999999999996270, 2.500000000000000000, 2.265063509461097357 ) ) ;
#80256=DIRECTION ( 'NONE',  ( -0.000000000000000000, -1.000000000000000000, -0.000000000000000000 ) ) ;
#80257=CARTESIAN_POINT ( 'NONE',  ( -14.14999999999998792, 2.500000000000000000, -1.572243186433547990 ) ) ;
#80258=ORIENTED_EDGE ( 'NONE', *, *, #43784, .T. ) ;
#80259=DIRECTION ( 'NONE',  ( 0.000000000000000000, 0.000000000000000000, 1.000000000000000000 ) ) ;
#80260=DIRECTION ( 'NONE',  ( 0.000000000000000000, 0.000000000000000000, 1.000000000000000000 ) ) ;
#80261=VERTEX_POINT ( 'NONE', #7442 ) ;
#80262=ORIENTED_EDGE ( 'NONE', *, *, #46912, .F. ) ;
#80263=VECTOR ( 'NONE', #93444, 1000.000000000000000 ) ;
#80264=AXIS2_PLACEMENT_3D ( 'NONE', #71323, #121719, #83106 ) ;
#80265=ORIENTED_EDGE ( 'NONE', *, *, #22881, .T. ) ;
#80266=LINE ( 'NONE', #58687, #31145 ) ;
#80267=CARTESIAN_POINT ( 'NONE',  ( -1.250000000000037526, 2.500000000000000000, -5.702370205355749455 ) ) ;
#80268=DIRECTION ( 'NONE',  ( 0.000000000000000000, 0.000000000000000000, -1.000000000000000000 ) ) ;
#80270=LINE ( 'NONE', #20066, #9329 ) ;
#80271=FACE_OUTER_BOUND ( 'NONE', #106789, .T. ) ;
#80272=CIRCLE ( 'NONE', #46819, 0.1000000000000002554 ) ;
#80273=AXIS2_PLACEMENT_3D ( 'NONE', #60644, #19395, #78995 ) ;
#80274=DIRECTION ( 'NONE',  ( 0.000000000000000000, -0.000000000000000000, 1.000000000000000000 ) ) ;
#80275=CARTESIAN_POINT ( 'NONE',  ( 7.949999999999925571, 12.50000000000000000, 2.230156782645134950 ) ) ;
#80276=CARTESIAN_POINT ( 'NONE',  ( -12.04999999999999716, 2.500000000000000000, -2.265063509461097802 ) ) ;
#80277=VECTOR ( 'NONE', #117888, 1000.000000000000000 ) ;
#80278=CIRCLE ( 'NONE', #74013, 0.1000000000000002554 ) ;
#80279=AXIS2_PLACEMENT_3D ( 'NONE', #116458, #13740, #55616 ) ;
#80280=VECTOR ( 'NONE', #41396, 1000.000000000000000 ) ;
#80281=ADVANCED_FACE ( 'NONE', ( #106927 ), #46741, .T. ) ;
#80282=ORIENTED_EDGE ( 'NONE', *, *, #12622, .T. ) ;
#80283=CARTESIAN_POINT ( 'NONE',  ( -0.6500000000000389910, 2.500000000000000000, -6.148780366869526226 ) ) ;
#80284=AXIS2_PLACEMENT_3D ( 'NONE', #46435, #77829, #126304 ) ;
#80285=EDGE_CURVE ( 'NONE', #106593, #73695, #107592, .T. ) ;
#80286=DIRECTION ( 'NONE',  ( -0.000000000000000000, -1.000000000000000000, -0.000000000000000000 ) ) ;
#80287=DIRECTION ( 'NONE',  ( 0.000000000000000000, 0.000000000000000000, 1.000000000000000000 ) ) ;
#80288=CARTESIAN_POINT ( 'NONE',  ( -11.05000000000000071, 2.500000000000000000, -6.841600689897075149 ) ) ;
#80289=LINE ( 'NONE', #120209, #100197 ) ;
#80290=EDGE_CURVE ( 'NONE', #109720, #115027, #113674, .T. ) ;
#80291=ORIENTED_EDGE ( 'NONE', *, *, #94645, .T. ) ;
#80292=CARTESIAN_POINT ( 'NONE',  ( 8.099999999999923261, 12.50000000000000000, 3.918623584224382839 ) ) ;
#80293=CARTESIAN_POINT ( 'NONE',  ( 3.099999999999945466, 12.50000000000000000, -3.983716857408426293 ) ) ;
#80294=CARTESIAN_POINT ( 'NONE',  ( 14.59999999999989484, 2.500000000000000000, 0.09999999999999772959 ) ) ;
#80295=ORIENTED_EDGE ( 'NONE', *, *, #60956, .F. ) ;
#80296=ADVANCED_FACE ( 'NONE', ( #58512 ), #107404, .T. ) ;
#80297=EDGE_CURVE ( 'NONE', #46288, #86969, #50993, .T. ) ;
#80298=EDGE_CURVE ( 'NONE', #56576, #21325, #38218, .T. ) ;
#80299=EDGE_CURVE ( 'NONE', #30852, #57931, #97361, .T. ) ;
#80300=EDGE_CURVE ( 'NONE', #53342, #112224, #88596, .T. ) ;
#80301=CIRCLE ( 'NONE', #19655, 0.1000000000000000056 ) ;
#80302=VERTEX_POINT ( 'NONE', #29047 ) ;
#80303=CARTESIAN_POINT ( 'NONE',  ( 14.14999999999989555, 2.500000000000000000, 2.065063509461097624 ) ) ;
#80304=ORIENTED_EDGE ( 'NONE', *, *, #52680, .F. ) ;
#80305=ORIENTED_EDGE ( 'NONE', *, *, #48450, .T. ) ;
#80306=CARTESIAN_POINT ( 'NONE',  ( 8.349999999999923261, 2.500000000000000000, -6.395190528383301931 ) ) ;
#80307=EDGE_CURVE ( 'NONE', #89533, #75765, #17944, .T. ) ;
#80308=CARTESIAN_POINT ( 'NONE',  ( 18.98912670146724579, 2.543039972613466482, -4.488908218019479257 ) ) ;
#80309=DIRECTION ( 'NONE',  ( 0.000000000000000000, -0.000000000000000000, 1.000000000000000000 ) ) ;
#80310=AXIS2_PLACEMENT_3D ( 'NONE', #31264, #39163, #36731 ) ;
#80312=CIRCLE ( 'NONE', #55175, 0.1000000000000002554 ) ;
#80313=EDGE_CURVE ( 'NONE', #115346, #70210, #34605, .T. ) ;
#80314=ORIENTED_EDGE ( 'NONE', *, *, #76888, .T. ) ;
#80315=DIRECTION ( 'NONE',  ( 0.000000000000000000, -0.000000000000000000, 1.000000000000000000 ) ) ;
#80316=ORIENTED_EDGE ( 'NONE', *, *, #96378, .T. ) ;
#80317=CARTESIAN_POINT ( 'NONE',  ( 0.8499999999999545697, 2.500000000000000000, 2.857883832488649301 ) ) ;
#80318=CARTESIAN_POINT ( 'NONE',  ( 17.17276927100807526, 1.352216491748947202, 5.266219974090748934 ) ) ;
#80319=CARTESIAN_POINT ( 'NONE',  ( -1.650000000000034328, 12.50000000000000000, -2.165063509461101710 ) ) ;
#80321=AXIS2_PLACEMENT_3D ( 'NONE', #20578, #2202, #60520 ) ;
#80322=VERTEX_POINT ( 'NONE', #55904 ) ;
#80323=ORIENTED_EDGE ( 'NONE', *, *, #93907, .F. ) ;
#80324=ORIENTED_EDGE ( 'NONE', *, *, #109861, .F. ) ;
#80325=ORIENTED_EDGE ( 'NONE', *, *, #104369, .T. ) ;
#80326=CARTESIAN_POINT ( 'NONE',  ( 11.64999999999990621, 12.50000000000000000, -2.099970236277064473 ) ) ;
#80327=CARTESIAN_POINT ( 'NONE',  ( 12.07106445316774135, 2.500000000000126121, 8.629160867384618072 ) ) ;
#80328=LINE ( 'NONE', #97376, #85842 ) ;
#80329=FACE_BOUND ( 'NONE', #62043, .T. ) ;
#80330=CARTESIAN_POINT ( 'NONE',  ( 10.59999999999990905, 2.500000000000000000, -4.083716857408426826 ) ) ;
#80332=CARTESIAN_POINT ( 'NONE',  ( 9.149999999999915090, 2.500000000000000000, -2.165063509461101710 ) ) ;
#80333=CARTESIAN_POINT ( 'NONE',  ( -6.850000000000013856, 12.50000000000000000, 6.083687093685483660 ) ) ;
#80334=AXIS2_PLACEMENT_3D ( 'NONE', #2708, #72118, #11889 ) ;
#80335=AXIS2_PLACEMENT_3D ( 'NONE', #62933, #60996, #2066 ) ;
#80336=DIRECTION ( 'NONE',  ( 0.000000000000000000, 0.000000000000000000, 1.000000000000000000 ) ) ;
#80337=EDGE_CURVE ( 'NONE', #76614, #23241, #6150, .T. ) ;
#80338=DIRECTION ( 'NONE',  ( 0.000000000000000000, 0.000000000000000000, -1.000000000000000000 ) ) ;
#80339=EDGE_CURVE ( 'NONE', #82216, #28777, #17243, .T. ) ;
#80340=DIRECTION ( 'NONE',  ( -4.274815082592931898E-19, -0.9999939076577903929, -0.003490651415223739937 ) ) ;
#80342=DIRECTION ( 'NONE',  ( 0.000000000000000000, 0.000000000000000000, -1.000000000000000000 ) ) ;
#80343=EDGE_CURVE ( 'NONE', #29645, #29366, #97123, .T. ) ;
#80344=EDGE_LOOP ( 'NONE', ( #46247, #77960, #13223, #119661 ) ) ;
#80345=EDGE_LOOP ( 'NONE', ( #1593, #11117 ) ) ;
#80346=ORIENTED_EDGE ( 'NONE', *, *, #25022, .F. ) ;
#80347=ORIENTED_EDGE ( 'NONE', *, *, #8048, .F. ) ;
#80348=CARTESIAN_POINT ( 'NONE',  ( -11.89999999999999680, 2.500000000000000000, 0.2464101615137776757 ) ) ;
#80349=DIRECTION ( 'NONE',  ( 0.000000000000000000, 1.000000000000000000, 0.000000000000000000 ) ) ;
#80350=ADVANCED_FACE ( 'NONE', ( #77480 ), #99440, .T. ) ;
#80351=FACE_BOUND ( 'NONE', #415, .T. ) ;
#80352=DIRECTION ( 'NONE',  ( 0.000000000000000000, 0.000000000000000000, 1.000000000000000000 ) ) ;
#80353=EDGE_CURVE ( 'NONE', #129332, #89461, #76439, .T. ) ;
#80354=EDGE_CURVE ( 'NONE', #126313, #59594, #51904, .T. ) ;
#80355=AXIS2_PLACEMENT_3D ( 'NONE', #19729, #119850, #60314 ) ;
#80356=AXIS2_PLACEMENT_3D ( 'NONE', #21495, #61441, #104563 ) ;
#80358=ORIENTED_EDGE ( 'NONE', *, *, #11310, .F. ) ;
#80359=CARTESIAN_POINT ( 'NONE',  ( -9.600000000000006750, 2.500000000000000000, 3.637306695894644726 ) ) ;
#80360=CIRCLE ( 'NONE', #40666, 0.06509327318403745899 ) ;
#80361=CARTESIAN_POINT ( 'NONE',  ( 11.89999999999990443, 2.500000000000000000, -0.3464101615137782364 ) ) ;
#80362=DIRECTION ( 'NONE',  ( -0.000000000000000000, -1.000000000000000000, -0.000000000000000000 ) ) ;
#80363=PLANE ( 'NONE',  #62088 ) ;
#80364=VERTEX_POINT ( 'NONE', #121924 ) ;
#80366=EDGE_CURVE ( 'NONE', #103956, #20627, #21136, .T. ) ;
#80367=CONICAL_SURFACE ( 'NONE', #21786, 0.1000000000000002554, 0.003490658503988666988 ) ;
#80368=AXIS2_PLACEMENT_3D ( 'NONE', #52874, #43720, #61424 ) ;
#80369=AXIS2_PLACEMENT_3D ( 'NONE', #32342, #102978, #35548 ) ;
#80370=ORIENTED_EDGE ( 'NONE', *, *, #58709, .T. ) ;
#80371=EDGE_LOOP ( 'NONE', ( #48321, #123940, #15518, #115143 ) ) ;
#80372=FACE_OUTER_BOUND ( 'NONE', #50114, .T. ) ;
#80373=DIRECTION ( 'NONE',  ( -0.000000000000000000, 1.000000000000000000, -0.000000000000000000 ) ) ;
#80374=ORIENTED_EDGE ( 'NONE', *, *, #324, .F. ) ;
#80375=VECTOR ( 'NONE', #79767, 1000.000000000000000 ) ;
#80376=CIRCLE ( 'NONE', #944, 0.09999999999999982514 ) ;
#80377=CARTESIAN_POINT ( 'NONE',  ( -9.800000000000007816, 2.500000000000000000, -4.083716857408422385 ) ) ;
#80378=FACE_OUTER_BOUND ( 'NONE', #8494, .T. ) ;
#80379=DIRECTION ( 'NONE',  ( 0.000000000000000000, 0.000000000000000000, 1.000000000000000000 ) ) ;
#80380=CONICAL_SURFACE ( 'NONE', #53198, 0.1000000000000002554, 0.003490658503988666988 ) ;
#80381=EDGE_LOOP ( 'NONE', ( #93236, #46378, #73412, #88898 ) ) ;
#80382=CARTESIAN_POINT ( 'NONE',  ( 3.349999999999945466, 12.50000000000000000, -7.188010851410854052 ) ) ;
#80383=EDGE_CURVE ( 'NONE', #127915, #47419, #111441, .T. ) ;
#80384=VERTEX_POINT ( 'NONE', #2140 ) ;
#80385=DIRECTION ( 'NONE',  ( 0.000000000000000000, -0.9999939076577903929, 0.003490651415223739937 ) ) ;
#80386=VERTEX_POINT ( 'NONE', #10646 ) ;
#80387=DIRECTION ( 'NONE',  ( 0.000000000000000000, 1.000000000000000000, 0.000000000000000000 ) ) ;
#80388=ORIENTED_EDGE ( 'NONE', *, *, #105921, .F. ) ;
#80389=DIRECTION ( 'NONE',  ( -0.000000000000000000, -1.000000000000000000, -0.000000000000000000 ) ) ;
#80390=CARTESIAN_POINT ( 'NONE',  ( -2.500000000000032863, 2.500000000000000000, 5.122947341949749323 ) ) ;
#80391=( BOUNDED_SURFACE ( )  B_SPLINE_SURFACE ( 3, 2, ( 
 ( #120429, #75191, #43175 ),
 ( #92916, #115748, #115086 ),
 ( #25423, #3237, #43818 ),
 ( #83090, #13019, #114464 ),
 ( #123007, #105297, #93542 ),
 ( #14941, #64718, #26101 ),
 ( #113172, #73256, #65353 ),
 ( #94829, #124935, #15609 ),
 ( #33358, #23503, #75822 ),
 ( #54896, #4484, #63439 ),
 ( #104636, #103369, #5149 ),
 ( #33981, #24805, #45100 ) ),
 .UNSPECIFIED., .F., .F., .F. ) 
 B_SPLINE_SURFACE_WITH_KNOTS ( ( 4, 2, 2, 2, 2, 4 ),
 ( 3, 3 ),
 ( -5.075233897202870062E-05, 0.01652955890749032222, 0.03310987015395267657, 0.04969018140041503440, 0.05798033702364620984, 0.06627049264687738528 ),
 ( 0.000000000000000000, 1.000000000000000000 ),
 .UNSPECIFIED. ) 
 GEOMETRIC_REPRESENTATION_ITEM ( )  RATIONAL_B_SPLINE_SURFACE ( (
 ( 1.000000000000000000, 1.000000000000000000, 1.000000000000000000),
 ( 1.000000000000000000, 0.9999962913217402827, 1.000000000000000000),
 ( 1.000000000000000000, 0.9967432547753130034, 1.000000000000000000),
 ( 1.000000000000000000, 0.9780629203681809880, 1.000000000000000000),
 ( 1.000000000000000000, 0.9624374449453717562, 1.000000000000000000),
 ( 1.000000000000000000, 0.9156028756800554946, 1.000000000000000000),
 ( 1.000000000000000000, 0.8842425818992938336, 1.000000000000000000),
 ( 1.000000000000000000, 0.8293059173961181418, 1.000000000000000000),
 ( 1.000000000000000000, 0.8097380764746227033, 1.000000000000000000),
 ( 1.000000000000000000, 0.7702514575415626563, 1.000000000000000000),
 ( 1.000000000000000000, 0.7503390841280456192, 1.000000000000000000),
 ( 1.000000000000000000, 0.7318752858502178826, 1.000000000000000000) ) ) 
 REPRESENTATION_ITEM ( '' )  SURFACE ( )  );
#80392=FACE_OUTER_BOUND ( 'NONE', #127042, .T. ) ;
#80393=FACE_OUTER_BOUND ( 'NONE', #111706, .T. ) ;
#80394=LINE ( 'NONE', #103890, #126874 ) ;
#80396=EDGE_LOOP ( 'NONE', ( #11591, #85669 ) ) ;
#80397=ORIENTED_EDGE ( 'NONE', *, *, #123031, .F. ) ;
#80398=DIRECTION ( 'NONE',  ( 0.000000000000000000, 1.000000000000000000, 0.000000000000000000 ) ) ;
#80399=ADVANCED_FACE ( 'NONE', ( #61734 ), #20013, .T. ) ;
#80400=DIRECTION ( 'NONE',  ( 0.000000000000000000, 1.000000000000000000, 0.000000000000000000 ) ) ;
#80401=DIRECTION ( 'NONE',  ( 0.000000000000000000, 0.000000000000000000, -1.000000000000000000 ) ) ;
#80402=VERTEX_POINT ( 'NONE', #81369 ) ;
#80403=ORIENTED_EDGE ( 'NONE', *, *, #129392, .T. ) ;
#80404=ORIENTED_EDGE ( 'NONE', *, *, #31835, .T. ) ;
#80405=DIRECTION ( 'NONE',  ( -0.000000000000000000, -1.000000000000000000, -0.000000000000000000 ) ) ;
#80406=CIRCLE ( 'NONE', #13475, 0.06509327318403745899 ) ;
#80407=EDGE_LOOP ( 'NONE', ( #35932, #14022, #44577, #103972 ) ) ;
#80408=CARTESIAN_POINT ( 'NONE',  ( 2.899999999999946620, 2.500000000000000000, -3.737306695894649700 ) ) ;
#80409=CIRCLE ( 'NONE', #53220, 0.06509327318403745899 ) ;
#80410=CARTESIAN_POINT ( 'NONE',  ( 10.84999999999991260, 2.500000000000000000, 7.088010851410848190 ) ) ;
#80411=DIRECTION ( 'NONE',  ( 0.000000000000000000, -0.9999939076577903929, 0.003490651415223739937 ) ) ;
#80412=DIRECTION ( 'NONE',  ( 0.000000000000000000, 1.000000000000000000, 0.000000000000000000 ) ) ;
#80413=DIRECTION ( 'NONE',  ( 0.000000000000000000, 0.000000000000000000, -1.000000000000000000 ) ) ;
#80414=CARTESIAN_POINT ( 'NONE',  ( 13.29999999999990301, 12.50000000000000000, 4.330127018922196314 ) ) ;
#80415=EDGE_CURVE ( 'NONE', #122496, #93275, #28325, .T. ) ;
#80416=DIRECTION ( 'NONE',  ( 0.000000000000000000, -0.9999939076577903929, 0.003490651415223739937 ) ) ;
#80417=VERTEX_POINT ( 'NONE', #72192 ) ;
#80418=EDGE_LOOP ( 'NONE', ( #65652, #91004 ) ) ;
#80419=AXIS2_PLACEMENT_3D ( 'NONE', #82735, #74831, #122641 ) ;
#80420=DIRECTION ( 'NONE',  ( -4.274815082592931898E-19, -0.9999939076577903929, -0.003490651415223739937 ) ) ;
#80421=DIRECTION ( 'NONE',  ( 0.000000000000000000, 1.000000000000000000, 0.000000000000000000 ) ) ;
#80422=AXIS2_PLACEMENT_3D ( 'NONE', #106099, #4641, #66799 ) ;
#80423=ORIENTED_EDGE ( 'NONE', *, *, #100529, .F. ) ;
#80424=ORIENTED_EDGE ( 'NONE', *, *, #72486, .T. ) ;
#80426=CARTESIAN_POINT ( 'NONE',  ( 5.649999999999936406, 12.50000000000000000, -6.213873640053564351 ) ) ;
#80427=FACE_OUTER_BOUND ( 'NONE', #88912, .T. ) ;
#80428=CARTESIAN_POINT ( 'NONE',  ( 4.599999999999940137, 2.500000000000000000, -5.022947341949754119 ) ) ;
#80429=CIRCLE ( 'NONE', #126388, 0.1000000000000002554 ) ;
#80430=DIRECTION ( 'NONE',  ( 0.000000000000000000, 0.000000000000000000, 1.000000000000000000 ) ) ;
#80431=CIRCLE ( 'NONE', #55289, 0.06509327318403745899 ) ;
#80432=CARTESIAN_POINT ( 'NONE',  ( 5.449999999999936229, 12.50000000000000000, 6.495190528383297135 ) ) ;
#80433=FACE_OUTER_BOUND ( 'NONE', #32297, .T. ) ;
#80434=CIRCLE ( 'NONE', #99216, 0.1000000000000000056 ) ;
#80435=CARTESIAN_POINT ( 'NONE',  ( 10.84999999999991260, 2.500000000000000000, 6.595190528383296780 ) ) ;
#80436=EDGE_LOOP ( 'NONE', ( #64690, #72580 ) ) ;
#80437=ORIENTED_EDGE ( 'NONE', *, *, #104937, .T. ) ;
#80438=EDGE_CURVE ( 'NONE', #89530, #121486, #36739, .T. ) ;
#80439=ORIENTED_EDGE ( 'NONE', *, *, #25209, .F. ) ;
#80440=VERTEX_POINT ( 'NONE', #21805 ) ;
#80441=ORIENTED_EDGE ( 'NONE', *, *, #30355, .T. ) ;
#80442=DIRECTION ( 'NONE',  ( 0.000000000000000000, -0.000000000000000000, 1.000000000000000000 ) ) ;
#80443=CARTESIAN_POINT ( 'NONE',  ( 2.899999999999944844, 12.50000000000000000, 3.702399969078682407 ) ) ;
#80444=ADVANCED_FACE ( 'NONE', ( #20509 ), #40960, .T. ) ;
#80445=ORIENTED_EDGE ( 'NONE', *, *, #53577, .F. ) ;
#80446=CARTESIAN_POINT ( 'NONE',  ( 11.89999999999990798, 2.500000000000000000, 3.983716857408420964 ) ) ;
#80447=CARTESIAN_POINT ( 'NONE',  ( 6.699999999999930012, 2.500000000000000000, 4.330127018922196314 ) ) ;
#80448=AXIS2_PLACEMENT_3D ( 'NONE', #41165, #20214, #19565 ) ;
#80449=CONICAL_SURFACE ( 'NONE', #34486, 0.1000000000000002554, 0.003490658503988666988 ) ;
#80450=CARTESIAN_POINT ( 'NONE',  ( 12.49999999999990230, 2.500000000000000000, -0.5928203230275541635 ) ) ;
#80451=DIRECTION ( 'NONE',  ( -0.000000000000000000, 1.000000000000000000, -0.000000000000000000 ) ) ;
#80452=ORIENTED_EDGE ( 'NONE', *, *, #100391, .T. ) ;
#80453=AXIS2_PLACEMENT_3D ( 'NONE', #14059, #24546, #95869 ) ;
#80454=ADVANCED_FACE ( 'NONE', ( #70248 ), #119335, .T. ) ;
#80455=CONICAL_SURFACE ( 'NONE', #34489, 0.1000000000000002554, 0.003490658503988666988 ) ;
#80457=EDGE_CURVE ( 'NONE', #85577, #70277, #7471, .T. ) ;
#80458=DIRECTION ( 'NONE',  ( 0.000000000000000000, 1.000000000000000000, 0.000000000000000000 ) ) ;
#80459=EDGE_CURVE ( 'NONE', #62448, #59275, #126624, .T. ) ;
#80460=FACE_OUTER_BOUND ( 'NONE', #9023, .T. ) ;
#80461=ORIENTED_EDGE ( 'NONE', *, *, #23445, .F. ) ;
#80462=AXIS2_PLACEMENT_3D ( 'NONE', #120654, #101007, #41473 ) ;
#80463=CONICAL_SURFACE ( 'NONE', #28310, 0.09999999999999982514, 0.003490658503988666988 ) ;
#80464=CONICAL_SURFACE ( 'NONE', #32455, 0.09999999999999982514, 0.003490658503988666988 ) ;
#80465=EDGE_CURVE ( 'NONE', #93446, #60636, #86891, .T. ) ;
#80466=VERTEX_POINT ( 'NONE', #59814 ) ;
#80467=EDGE_CURVE ( 'NONE', #97708, #93625, #11588, .T. ) ;
#80468=ORIENTED_EDGE ( 'NONE', *, *, #46757, .T. ) ;
#80469=EDGE_LOOP ( 'NONE', ( #16822, #115106 ) ) ;
#80470=FACE_OUTER_BOUND ( 'NONE', #57915, .T. ) ;
#80471=CONICAL_SURFACE ( 'NONE', #78417, 0.1000000000000002554, 0.003490658503988666988 ) ;
#80472=ADVANCED_FACE ( 'NONE', ( #120633 ), #120363, .T. ) ;
#80473=DIRECTION ( 'NONE',  ( 0.000000000000000000, -0.9999939076577903929, 0.003490651415223739937 ) ) ;
#80474=DIRECTION ( 'NONE',  ( 0.000000000000000000, 0.000000000000000000, 1.000000000000000000 ) ) ;
#80475=EDGE_CURVE ( 'NONE', #72217, #74701, #45061, .T. ) ;
#80476=AXIS2_PLACEMENT_3D ( 'NONE', #115007, #56095, #33269 ) ;
#80477=AXIS2_PLACEMENT_3D ( 'NONE', #55249, #45431, #55876 ) ;
#80478=ADVANCED_FACE ( 'NONE', ( #119994 ), #110176, .T. ) ;
#80479=CARTESIAN_POINT ( 'NONE',  ( 3.749999999999942268, 2.500000000000000000, -1.372243186433550033 ) ) ;
#80480=CIRCLE ( 'NONE', #40776, 0.09999999999999982514 ) ;
#80481=EDGE_LOOP ( 'NONE', ( #286, #40010, #47270, #127189 ) ) ;
#80482=CARTESIAN_POINT ( 'NONE',  ( -5.650000000000019895, 2.500000000000000000, 6.148780366869520009 ) ) ;
#80483=CARTESIAN_POINT ( 'NONE',  ( 16.86635082839119804, -0.4716143926291150867, -5.778906370536186721 ) ) ;
#80484=CARTESIAN_POINT ( 'NONE',  ( 4.349999999999941025, 12.50000000000000000, -6.213873640053564351 ) ) ;
#80485=DIRECTION ( 'NONE',  ( -0.000000000000000000, -1.000000000000000000, -0.000000000000000000 ) ) ;
#80487=ORIENTED_EDGE ( 'NONE', *, *, #86348, .T. ) ;
#80488=DIRECTION ( 'NONE',  ( -0.000000000000000000, -1.000000000000000000, -0.000000000000000000 ) ) ;
#80489=EDGE_LOOP ( 'NONE', ( #116284, #124517 ) ) ;
#80490=ORIENTED_EDGE ( 'NONE', *, *, #109078, .T. ) ;
#80491=DIRECTION ( 'NONE',  ( 0.000000000000000000, 1.000000000000000000, 0.000000000000000000 ) ) ;
#80492=DIRECTION ( 'NONE',  ( -0.000000000000000000, 1.000000000000000000, -0.000000000000000000 ) ) ;
#80493=FACE_BOUND ( 'NONE', #120042, .T. ) ;
#80494=CARTESIAN_POINT ( 'NONE',  ( -14.54999999999998472, 2.500000000000000000, -2.165063509461099489 ) ) ;
#80495=DIRECTION ( 'NONE',  ( -0.000000000000000000, 1.000000000000000000, -0.000000000000000000 ) ) ;
#80496=DIRECTION ( 'NONE',  ( -4.274815082592931898E-19, -0.9999939076577903929, -0.003490651415223739937 ) ) ;
#80497=CARTESIAN_POINT ( 'NONE',  ( 9.149999999999918643, 12.50000000000000000, -6.560283801567339701 ) ) ;
#80498=ADVANCED_FACE ( 'NONE', ( #34198 ), #45307, .T. ) ;
#80499=CARTESIAN_POINT ( 'NONE',  ( 11.84999999999990372, 12.50000000000000000, -6.906693963081115939 ) ) ;
#80500=DIRECTION ( 'NONE',  ( 0.000000000000000000, -0.000000000000000000, 1.000000000000000000 ) ) ;
#80501=CARTESIAN_POINT ( 'NONE',  ( 12.29999999999990479, 2.500000000000000000, -3.883716857408426648 ) ) ;
#80502=VERTEX_POINT ( 'NONE', #104840 ) ;
#80503=AXIS2_PLACEMENT_3D ( 'NONE', #54876, #46347, #115073 ) ;
#80504=DIRECTION ( 'NONE',  ( 0.000000000000000000, 0.000000000000000000, -1.000000000000000000 ) ) ;
#80505=CARTESIAN_POINT ( 'NONE',  ( -6.250000000000015987, 2.500000000000000000, 1.572243186433545548 ) ) ;
#80506=ORIENTED_EDGE ( 'NONE', *, *, #101028, .T. ) ;
#80507=VERTEX_POINT ( 'NONE', #74119 ) ;
#80508=DIRECTION ( 'NONE',  ( -0.000000000000000000, 1.000000000000000000, -0.000000000000000000 ) ) ;
#80509=DIRECTION ( 'NONE',  ( 0.000000000000000000, 1.000000000000000000, 0.000000000000000000 ) ) ;
#80510=FACE_BOUND ( 'NONE', #27716, .T. ) ;
#80511=DIRECTION ( 'NONE',  ( 0.000000000000000000, 0.000000000000000000, -1.000000000000000000 ) ) ;
#80512=CIRCLE ( 'NONE', #59688, 0.1000000000000002554 ) ;
#80513=EDGE_CURVE ( 'NONE', #15869, #46460, #94381, .T. ) ;
#80514=CARTESIAN_POINT ( 'NONE',  ( -10.40000000000000213, 2.500000000000000000, -4.330127018922197202 ) ) ;
#80515=CIRCLE ( 'NONE', #13585, 0.06509327318403745899 ) ;
#80516=EDGE_CURVE ( 'NONE', #91809, #21509, #91104, .T. ) ;
#80517=ORIENTED_EDGE ( 'NONE', *, *, #112839, .F. ) ;
#80518=CARTESIAN_POINT ( 'NONE',  ( -2.700000000000029932, 2.500000000000000000, -4.776537180435977525 ) ) ;
#80519=ORIENTED_EDGE ( 'NONE', *, *, #15701, .F. ) ;
#80520=DIRECTION ( 'NONE',  ( 0.000000000000000000, 0.000000000000000000, 1.000000000000000000 ) ) ;
#80521=DIRECTION ( 'NONE',  ( 0.000000000000000000, -0.000000000000000000, 1.000000000000000000 ) ) ;
#80522=EDGE_CURVE ( 'NONE', #40128, #96204, #12595, .T. ) ;
#80523=VECTOR ( 'NONE', #78254, 1000.000000000000000 ) ;
#80524=CIRCLE ( 'NONE', #42888, 0.06509327318403745899 ) ;
#80525=DIRECTION ( 'NONE',  ( 0.000000000000000000, 0.000000000000000000, 1.000000000000000000 ) ) ;
#80526=PLANE ( 'NONE',  #19596 ) ;
#80527=ORIENTED_EDGE ( 'NONE', *, *, #95401, .T. ) ;
#80528=CARTESIAN_POINT ( 'NONE',  ( 4.349999999999936584, 2.500000000000000000, 6.148780366869520009 ) ) ;
#80529=DIRECTION ( 'NONE',  ( 0.000000000000000000, -0.000000000000000000, 1.000000000000000000 ) ) ;
#80531=VERTEX_POINT ( 'NONE', #64282 ) ;
#80532=EDGE_LOOP ( 'NONE', ( #60952, #67515, #118479, #76620 ) ) ;
#80533=DIRECTION ( 'NONE',  ( 0.000000000000000000, 0.000000000000000000, 1.000000000000000000 ) ) ;
#80534=EDGE_LOOP ( 'NONE', ( #90847, #116106, #81724, #102793 ) ) ;
#80535=CARTESIAN_POINT ( 'NONE',  ( 11.89999999999990443, 12.50000000000000000, 0.2813168883297362810 ) ) ;
#80536=CARTESIAN_POINT ( 'NONE',  ( 87.50000000000000000, -7.402262750143061787, 1.385127402881718650 ) ) ;
#80537=AXIS2_PLACEMENT_3D ( 'NONE', #82791, #104345, #93884 ) ;
#80538=DIRECTION ( 'NONE',  ( -0.000000000000000000, 1.000000000000000000, -0.000000000000000000 ) ) ;
#80539=EDGE_LOOP ( 'NONE', ( #53310, #10048 ) ) ;
#80540=CIRCLE ( 'NONE', #68002, 0.1000000000000002554 ) ;
#80541=DIRECTION ( 'NONE',  ( -4.274815082592931898E-19, -0.9999939076577903929, -0.003490651415223739937 ) ) ;
#80542=DIRECTION ( 'NONE',  ( 0.000000000000000000, 0.000000000000000000, -1.000000000000000000 ) ) ;
#80543=CARTESIAN_POINT ( 'NONE',  ( -9.999999999999971578, 2.500000000000000000, -4.330127018922197202 ) ) ;
#80544=CIRCLE ( 'NONE', #120252, 0.06509327318403745899 ) ;
#80545=DIRECTION ( 'NONE',  ( 0.000000000000000000, -0.9999939076577903929, 0.003490651415223739937 ) ) ;
#80546=CARTESIAN_POINT ( 'NONE',  ( 3.349999999999942801, 12.50000000000000000, 2.857883832488649301 ) ) ;
#80547=CARTESIAN_POINT ( 'NONE',  ( -0.8500000000000386136, 12.50000000000000000, 5.867463478539781896 ) ) ;
#80548=ORIENTED_EDGE ( 'NONE', *, *, #3207, .F. ) ;
#80549=ORIENTED_EDGE ( 'NONE', *, *, #38814, .F. ) ;
#80551=CARTESIAN_POINT ( 'NONE',  ( 10.84999999999991260, 2.500000000000000000, -1.472243186433550122 ) ) ;
#80552=VERTEX_POINT ( 'NONE', #53821 ) ;
#80554=AXIS2_PLACEMENT_3D ( 'NONE', #26521, #86059, #17310 ) ;
#80555=ORIENTED_EDGE ( 'NONE', *, *, #110778, .F. ) ;
#80557=ORIENTED_EDGE ( 'NONE', *, *, #127023, .T. ) ;
#80558=CARTESIAN_POINT ( 'NONE',  ( -5.650000000000023448, 12.50000000000000000, -6.148780366869526226 ) ) ;
#80559=FACE_OUTER_BOUND ( 'NONE', #49302, .T. ) ;
#80560=CONICAL_SURFACE ( 'NONE', #26264, 0.1000000000000000472, 0.003490658503988666988 ) ;
#80561=DIRECTION ( 'NONE',  ( 0.000000000000000000, -0.000000000000000000, 1.000000000000000000 ) ) ;
#80563=LINE ( 'NONE', #90355, #109979 ) ;
#80564=CARTESIAN_POINT ( 'NONE',  ( 0.000000000000000000, -2.500000000000000000, 0.000000000000000000 ) ) ;
#80566=AXIS2_PLACEMENT_3D ( 'NONE', #117929, #7974, #87815 ) ;
#80567=EDGE_CURVE ( 'NONE', #62966, #82761, #49265, .T. ) ;
#80568=FACE_OUTER_BOUND ( 'NONE', #77953, .T. ) ;
#80569=DIRECTION ( 'NONE',  ( -4.274815082592931898E-19, -0.9999939076577903929, -0.003490651415223739937 ) ) ;
#80570=ADVANCED_FACE ( 'NONE', ( #104209 ), #95227, .T. ) ;
#80571=DIRECTION ( 'NONE',  ( 0.000000000000000000, 1.000000000000000000, 0.000000000000000000 ) ) ;
#80572=ORIENTED_EDGE ( 'NONE', *, *, #111809, .F. ) ;
#80573=CARTESIAN_POINT ( 'NONE',  ( 8.099999999999923261, 2.500000000000000000, -3.983716857408426293 ) ) ;
#80574=VERTEX_POINT ( 'NONE', #102914 ) ;
#80575=ADVANCED_FACE ( 'NONE', ( #13234 ), #122420, .T. ) ;
#80576=VERTEX_POINT ( 'NONE', #2788 ) ;
#80577=CARTESIAN_POINT ( 'NONE',  ( 9.349999999999916156, 2.500000000000000000, -1.918653347947326004 ) ) ;
#80578=AXIS2_PLACEMENT_3D ( 'NONE', #62962, #93713, #91779 ) ;
#80579=DIRECTION ( 'NONE',  ( -4.274815082592931898E-19, -0.9999939076577903929, -0.003490651415223739937 ) ) ;
#80580=CARTESIAN_POINT ( 'NONE',  ( 3.749999999999942268, 12.50000000000000000, -1.537336459617587581 ) ) ;
#80581=CARTESIAN_POINT ( 'NONE',  ( 13.74999999999989519, 2.500000000000000000, -2.857883832488653741 ) ) ;
#80582=CARTESIAN_POINT ( 'NONE',  ( -11.84999999999999787, 12.50000000000000000, -1.818653347947321919 ) ) ;
#80583=DIRECTION ( 'NONE',  ( 0.000000000000000000, -0.9999939076577903929, 0.003490651415223739937 ) ) ;
#80584=ORIENTED_EDGE ( 'NONE', *, *, #25745, .T. ) ;
#80585=AXIS2_PLACEMENT_3D ( 'NONE', #90480, #72161, #100326 ) ;
#80586=CIRCLE ( 'NONE', #118228, 0.1000000000000000056 ) ;
#80587=CIRCLE ( 'NONE', #111885, 0.06509327318403745899 ) ;
#80588=ORIENTED_EDGE ( 'NONE', *, *, #25019, .T. ) ;
#80589=DIRECTION ( 'NONE',  ( 0.000000000000000000, 1.000000000000000000, 0.000000000000000000 ) ) ;
#80590=ORIENTED_EDGE ( 'NONE', *, *, #19892, .T. ) ;
#80591=DIRECTION ( 'NONE',  ( -0.000000000000000000, -1.000000000000000000, -0.000000000000000000 ) ) ;
#80592=EDGE_CURVE ( 'NONE', #28605, #59465, #65968, .T. ) ;
#80593=ORIENTED_EDGE ( 'NONE', *, *, #119017, .T. ) ;
#80594=ORIENTED_EDGE ( 'NONE', *, *, #58775, .F. ) ;
#80595=DIRECTION ( 'NONE',  ( 0.000000000000000000, 0.000000000000000000, 1.000000000000000000 ) ) ;
#80596=LINE ( 'NONE', #79937, #12931 ) ;
#80597=CIRCLE ( 'NONE', #3316, 0.1000000000000002554 ) ;
#80598=EDGE_CURVE ( 'NONE', #57867, #68264, #32546, .T. ) ;
#80599=DIRECTION ( 'NONE',  ( 1.000000000000000000, 0.000000000000000000, 0.000000000000000000 ) ) ;
#80600=CARTESIAN_POINT ( 'NONE',  ( -11.25000000000000000, 12.50000000000000000, 7.188010851410848723 ) ) ;
#80601=CARTESIAN_POINT ( 'NONE',  ( 10.59999999999990905, 2.500000000000000000, -4.776537180435978414 ) ) ;
#80602=ORIENTED_EDGE ( 'NONE', *, *, #34209, .F. ) ;
#80603=CARTESIAN_POINT ( 'NONE',  ( -6.850000000000013856, 12.50000000000000000, 1.818653347947321475 ) ) ;
#80604=DIRECTION ( 'NONE',  ( -0.000000000000000000, -1.000000000000000000, -0.000000000000000000 ) ) ;
#80605=ADVANCED_FACE ( 'NONE', ( #102288 ), #3367, .T. ) ;
#80606=EDGE_CURVE ( 'NONE', #124839, #30668, #58385, .T. ) ;
#80607=DIRECTION ( 'NONE',  ( 0.000000000000000000, -0.000000000000000000, 1.000000000000000000 ) ) ;
#80608=EDGE_CURVE ( 'NONE', #106259, #5504, #38912, .T. ) ;
#80609=DIRECTION ( 'NONE',  ( 0.000000000000000000, 1.000000000000000000, 0.000000000000000000 ) ) ;
#80610=ADVANCED_FACE ( 'NONE', ( #43381 ), #99525, .T. ) ;
#80611=CARTESIAN_POINT ( 'NONE',  ( 1.049999999999952971, 12.50000000000000000, 6.148780366869520897 ) ) ;
#80612=ORIENTED_EDGE ( 'NONE', *, *, #25929, .T. ) ;
#80613=CIRCLE ( 'NONE', #24166, 0.06509327318403745899 ) ;
#80614=ORIENTED_EDGE ( 'NONE', *, *, #129330, .T. ) ;
#80615=ADVANCED_FACE ( 'NONE', ( #97611 ), #7554, .T. ) ;
#80616=DIRECTION ( 'NONE',  ( 0.000000000000000000, 0.000000000000000000, 1.000000000000000000 ) ) ;
#80617=EDGE_CURVE ( 'NONE', #63390, #79899, #28421, .T. ) ;
#80618=EDGE_LOOP ( 'NONE', ( #118321, #100585 ) ) ;
#80619=CARTESIAN_POINT ( 'NONE',  ( -8.950000000000011724, 12.50000000000000000, -6.148780366869520897 ) ) ;
#80620=CARTESIAN_POINT ( 'NONE',  ( -11.84999999999999609, 2.500000000000000000, 1.818653347947321475 ) ) ;
#80622=ADVANCED_FACE ( 'NONE', ( #116598 ), #107918, .T. ) ;
#80623=AXIS2_PLACEMENT_3D ( 'NONE', #40472, #29999, #10961 ) ;
#80624=ORIENTED_EDGE ( 'NONE', *, *, #11569, .T. ) ;
#80625=CARTESIAN_POINT ( 'NONE',  ( 4.799999999999935874, 2.500000000000000000, 3.983716857408420964 ) ) ;
#80626=DIRECTION ( 'NONE',  ( 0.000000000000000000, 0.000000000000000000, 1.000000000000000000 ) ) ;
#80627=EDGE_CURVE ( 'NONE', #87583, #120916, #47884, .T. ) ;
#80628=DIRECTION ( 'NONE',  ( -0.000000000000000000, 1.000000000000000000, -0.000000000000000000 ) ) ;
#80629=CIRCLE ( 'NONE', #40936, 0.06509327318403745899 ) ;
#80630=CARTESIAN_POINT ( 'NONE',  ( -1.250000000000001554, 12.50000000000000000, 2.165063509461097713 ) ) ;
#80631=EDGE_CURVE ( 'NONE', #92009, #15907, #43112, .T. ) ;
#80632=AXIS2_PLACEMENT_3D ( 'NONE', #7415, #25777, #66973 ) ;
#80633=DIRECTION ( 'NONE',  ( 0.000000000000000000, 1.000000000000000000, 0.000000000000000000 ) ) ;
#80634=CIRCLE ( 'NONE', #57643, 0.1000000000000000472 ) ;
#80635=VERTEX_POINT ( 'NONE', #88424 ) ;
#80636=CARTESIAN_POINT ( 'NONE',  ( 65.40766660093524365, 3.109053433052308968, -5.794607793964218878 ) ) ;
#80637=FACE_OUTER_BOUND ( 'NONE', #21451, .T. ) ;
#80638=CARTESIAN_POINT ( 'NONE',  ( -4.550000000000022915, 2.500000000000000000, -2.265063509461101798 ) ) ;
#80639=AXIS2_PLACEMENT_3D ( 'NONE', #75257, #123080, #74618 ) ;
#80640=DIRECTION ( 'NONE',  ( 0.000000000000000000, 1.000000000000000000, 0.000000000000000000 ) ) ;
#80641=EDGE_LOOP ( 'NONE', ( #98403, #69549, #87789, #54203 ) ) ;
#80642=CONICAL_SURFACE ( 'NONE', #66050, 0.09999999999999982514, 0.003490658503988666988 ) ;
#80643=EDGE_LOOP ( 'NONE', ( #18876, #117490 ) ) ;
#80644=CARTESIAN_POINT ( 'NONE',  ( -2.050000000000033129, 2.500000000000000000, 6.395190528383296602 ) ) ;
#80645=CARTESIAN_POINT ( 'NONE',  ( -2.300000000000032685, 12.50000000000000000, -4.676537180435978769 ) ) ;
#80646=DIRECTION ( 'NONE',  ( -0.000000000000000000, -1.000000000000000000, -0.000000000000000000 ) ) ;
#80647=ORIENTED_EDGE ( 'NONE', *, *, #101309, .F. ) ;
#80648=CONICAL_SURFACE ( 'NONE', #22174, 0.1000000000000000472, 0.003490658503988666988 ) ;
#80649=AXIS2_PLACEMENT_3D ( 'NONE', #96934, #24980, #95019 ) ;
#80650=CARTESIAN_POINT ( 'NONE',  ( -4.350000000000023626, 2.500000000000000000, -2.511473670974877948 ) ) ;
#80651=AXIS2_PLACEMENT_3D ( 'NONE', #1492, #49984, #71522 ) ;
#80652=FACE_OUTER_BOUND ( 'NONE', #97430, .T. ) ;
#80653=CIRCLE ( 'NONE', #24217, 0.1000000000000002554 ) ;
#80654=ORIENTED_EDGE ( 'NONE', *, *, #65212, .F. ) ;
#80655=CARTESIAN_POINT ( 'NONE',  ( 9.149999999999920419, 2.500000000000000000, 1.372243186433545370 ) ) ;
#80656=EDGE_LOOP ( 'NONE', ( #79798, #69104, #61715, #104642 ) ) ;
#80657=FACE_OUTER_BOUND ( 'NONE', #98162, .T. ) ;
#80658=EDGE_CURVE ( 'NONE', #113873, #59573, #30579, .T. ) ;
#80659=ORIENTED_EDGE ( 'NONE', *, *, #78409, .F. ) ;
#80660=CARTESIAN_POINT ( 'NONE',  ( 1.249999999999986899, 2.500000000000000000, 6.495190528383297135 ) ) ;
#80661=CARTESIAN_POINT ( 'NONE',  ( 12.89999999999990266, 2.500000000000000000, -3.637306695894650055 ) ) ;
#80662=EDGE_CURVE ( 'NONE', #28046, #34246, #78602, .T. ) ;
#80663=ORIENTED_EDGE ( 'NONE', *, *, #75879, .F. ) ;
#80664=VERTEX_POINT ( 'NONE', #76688 ) ;
#80666=CARTESIAN_POINT ( 'NONE',  ( -2.100000000000033396, 2.500000000000000000, 0.7928203230275495672 ) ) ;
#80667=AXIS2_PLACEMENT_3D ( 'NONE', #123641, #32731, #34000 ) ;
#80668=ORIENTED_EDGE ( 'NONE', *, *, #54109, .T. ) ;
#80669=DIRECTION ( 'NONE',  ( 0.000000000000000000, 0.000000000000000000, -1.000000000000000000 ) ) ;
#80670=LINE ( 'NONE', #20454, #93222 ) ;
#80671=DIRECTION ( 'NONE',  ( 0.000000000000000000, 0.000000000000000000, 1.000000000000000000 ) ) ;
#80673=DIRECTION ( 'NONE',  ( 0.000000000000000000, 1.000000000000000000, 0.000000000000000000 ) ) ;
#80674=CARTESIAN_POINT ( 'NONE',  ( 14.14999999999989555, 2.500000000000000000, 2.165063509461097713 ) ) ;
#80675=AXIS2_PLACEMENT_3D ( 'NONE', #117848, #109987, #91627 ) ;
#80676=CARTESIAN_POINT ( 'NONE',  ( 1.649999999999951950, 2.500000000000000000, -7.288010851410854585 ) ) ;
#80677=CIRCLE ( 'NONE', #9656, 0.06509327318403743123 ) ;
#80678=AXIS2_PLACEMENT_3D ( 'NONE', #71007, #112863, #61183 ) ;
#80680=AXIS2_PLACEMENT_3D ( 'NONE', #21576, #111219, #9178 ) ;
#80681=VERTEX_POINT ( 'NONE', #27562 ) ;
#80682=CARTESIAN_POINT ( 'NONE',  ( -2.500000000000030642, 12.50000000000000000, -4.957854068765716882 ) ) ;
#80683=ORIENTED_EDGE ( 'NONE', *, *, #113973, .F. ) ;
#80684=DIRECTION ( 'NONE',  ( 0.000000000000000000, 0.000000000000000000, 1.000000000000000000 ) ) ;
#80685=CARTESIAN_POINT ( 'NONE',  ( 7.499999999999923617, 12.50000000000000000, 0.6928203230275494784 ) ) ;
#80686=CARTESIAN_POINT ( 'NONE',  ( 8.099999999999923261, 12.50000000000000000, -3.983716857408426293 ) ) ;
#80687=EDGE_LOOP ( 'NONE', ( #14375, #118799 ) ) ;
#80688=ORIENTED_EDGE ( 'NONE', *, *, #68777, .F. ) ;
#80689=FACE_BOUND ( 'NONE', #107883, .T. ) ;
#80690=ORIENTED_EDGE ( 'NONE', *, *, #88253, .T. ) ;
#80691=DIRECTION ( 'NONE',  ( 0.000000000000000000, 0.000000000000000000, 1.000000000000000000 ) ) ;
#80692=CARTESIAN_POINT ( 'NONE',  ( 4.799999999999934097, 12.50000000000000000, 4.676537180435972552 ) ) ;
#80693=CIRCLE ( 'NONE', #72380, 0.1000000000000002554 ) ;
#80694=CARTESIAN_POINT ( 'NONE',  ( 7.299999999999927880, 12.50000000000000000, 3.918623584224383727 ) ) ;
#80695=LINE ( 'NONE', #126063, #120400 ) ;
#80696=CARTESIAN_POINT ( 'NONE',  ( 1.249999999999952038, 2.500000000000000000, 2.957883832488649389 ) ) ;
#80697=VECTOR ( 'NONE', #129029, 1000.000000000000000 ) ;
#80698=VECTOR ( 'NONE', #72164, 1000.000000000000000 ) ;
#80699=DIRECTION ( 'NONE',  ( 0.000000000000000000, 1.000000000000000000, 0.000000000000000000 ) ) ;
#80700=PLANE ( 'NONE',  #79000 ) ;
#80701=DIRECTION ( 'NONE',  ( 0.000000000000000000, -0.000000000000000000, 1.000000000000000000 ) ) ;
#80702=CARTESIAN_POINT ( 'NONE',  ( -11.64999999999999680, 12.50000000000000000, 2.230156782645134950 ) ) ;
#80703=CARTESIAN_POINT ( 'NONE',  ( 2.499999999999947153, 2.500000000000000000, 0.7928203230275495672 ) ) ;
#80704=EDGE_CURVE ( 'NONE', #87465, #11458, #49366, .T. ) ;
#80705=AXIS2_PLACEMENT_3D ( 'NONE', #7888, #109315, #9187 ) ;
#80706=ORIENTED_EDGE ( 'NONE', *, *, #127596, .F. ) ;
#80707=ORIENTED_EDGE ( 'NONE', *, *, #70117, .F. ) ;
#80708=AXIS2_PLACEMENT_3D ( 'NONE', #66822, #17720, #28860 ) ;
#80709=ORIENTED_EDGE ( 'NONE', *, *, #24281, .F. ) ;
#80710=ORIENTED_EDGE ( 'NONE', *, *, #15109, .T. ) ;
#80711=CARTESIAN_POINT ( 'NONE',  ( -3.950000000000029932, 12.50000000000000000, -6.213873640053564351 ) ) ;
#80712=PLANE ( 'NONE',  #105120 ) ;
#80713=ORIENTED_EDGE ( 'NONE', *, *, #18824, .T. ) ;
#80714=EDGE_LOOP ( 'NONE', ( #33195, #39070, #97402, #88980 ) ) ;
#80715=ORIENTED_EDGE ( 'NONE', *, *, #107933, .T. ) ;
#80716=CARTESIAN_POINT ( 'NONE',  ( -6.850000000000017408, 2.500000000000000000, -6.941600689897077459 ) ) ;
#80717=LINE ( 'NONE', #19860, #82243 ) ;
#80718=DIRECTION ( 'NONE',  ( 1.000000000000000000, 0.000000000000000000, 0.000000000000000000 ) ) ;
#80719=DIRECTION ( 'NONE',  ( -0.000000000000000000, 1.000000000000000000, -0.000000000000000000 ) ) ;
#80720=DIRECTION ( 'NONE',  ( -0.000000000000000000, 1.000000000000000000, -0.000000000000000000 ) ) ;
#80721=CARTESIAN_POINT ( 'NONE',  ( -8.100000000000013856, 2.500000000000000000, 0.4464101615137736623 ) ) ;
#80722=ADVANCED_FACE ( 'NONE', ( #107433 ), #68104, .T. ) ;
#80723=DIRECTION ( 'NONE',  ( 0.000000000000000000, 0.000000000000000000, 1.000000000000000000 ) ) ;
#80724=EDGE_CURVE ( 'NONE', #42654, #47060, #103731, .T. ) ;
#80725=ORIENTED_EDGE ( 'NONE', *, *, #25902, .F. ) ;
#80726=DIRECTION ( 'NONE',  ( -4.274815082592931898E-19, -0.9999939076577903929, -0.003490651415223739937 ) ) ;
#80727=VERTEX_POINT ( 'NONE', #17750 ) ;
#80728=VERTEX_POINT ( 'NONE', #66853 ) ;
#80729=EDGE_LOOP ( 'NONE', ( #62047, #120173, #26895, #78808 ) ) ;
#80730=AXIS2_PLACEMENT_3D ( 'NONE', #87179, #27608, #59029 ) ;
#80731=DIRECTION ( 'NONE',  ( -0.000000000000000000, -1.000000000000000000, -0.000000000000000000 ) ) ;
#80732=VERTEX_POINT ( 'NONE', #18408 ) ;
#80733=ADVANCED_FACE ( 'NONE', ( #58353 ), #98249, .T. ) ;
#80734=ORIENTED_EDGE ( 'NONE', *, *, #95102, .T. ) ;
#80735=ORIENTED_EDGE ( 'NONE', *, *, #103325, .T. ) ;
#80736=DIRECTION ( 'NONE',  ( 0.000000000000000000, 0.000000000000000000, 1.000000000000000000 ) ) ;
#80737=AXIS2_PLACEMENT_3D ( 'NONE', #23278, #103135, #114244 ) ;
#80738=AXIS2_PLACEMENT_3D ( 'NONE', #52162, #120892, #80342 ) ;
#80739=CARTESIAN_POINT ( 'NONE',  ( -10.85000000000000142, 2.500000000000000000, -7.088010851410849966 ) ) ;
#80740=CARTESIAN_POINT ( 'NONE',  ( 15.79999999999989058, 12.50000000000000000, -0.06509327318403980434 ) ) ;
#80741=DIRECTION ( 'NONE',  ( 0.000000000000000000, 0.000000000000000000, 1.000000000000000000 ) ) ;
#80742=DIRECTION ( 'NONE',  ( 0.000000000000000000, 0.000000000000000000, 1.000000000000000000 ) ) ;
#80743=FACE_OUTER_BOUND ( 'NONE', #66331, .T. ) ;
#80744=LINE ( 'NONE', #72216, #32537 ) ;
#80745=AXIS2_PLACEMENT_3D ( 'NONE', #17122, #57076, #47281 ) ;
#80746=EDGE_LOOP ( 'NONE', ( #42570, #98278, #85720, #124773 ) ) ;
#80747=DIRECTION ( 'NONE',  ( 0.000000000000000000, -0.9999939076577903929, 0.003490651415223739937 ) ) ;
#80748=CIRCLE ( 'NONE', #105774, 0.06509327318403745899 ) ;
#80749=EDGE_LOOP ( 'NONE', ( #34361, #117140, #39058, #27305 ) ) ;
#80751=CARTESIAN_POINT ( 'NONE',  ( 9.999999999999912959, 2.500000000000000000, -5.022947341949754119 ) ) ;
#80752=VERTEX_POINT ( 'NONE', #75380 ) ;
#80753=CARTESIAN_POINT ( 'NONE',  ( -0.2000000000000412836, 2.500000000000000000, 4.576537180435972019 ) ) ;
#80754=DIRECTION ( 'NONE',  ( 0.000000000000000000, 0.000000000000000000, 1.000000000000000000 ) ) ;
#80756=EDGE_CURVE ( 'NONE', #117090, #125178, #115287, .T. ) ;
#80757=DIRECTION ( 'NONE',  ( 0.000000000000000000, 0.000000000000000000, 1.000000000000000000 ) ) ;
#80758=EDGE_LOOP ( 'NONE', ( #7215, #60704 ) ) ;
#80759=EDGE_LOOP ( 'NONE', ( #96679, #90592 ) ) ;
#80760=CARTESIAN_POINT ( 'NONE',  ( 8.099999999999923261, 12.50000000000000000, -3.918623584224389056 ) ) ;
#80761=FACE_OUTER_BOUND ( 'NONE', #67045, .T. ) ;
#80762=ADVANCED_FACE ( 'NONE', ( #66209 ), #95310, .T. ) ;
#80764=CONICAL_SURFACE ( 'NONE', #24313, 0.1000000000000002554, 0.003490658503988666988 ) ;
#80765=CARTESIAN_POINT ( 'NONE',  ( -7.100000000000017408, 2.500000000000000000, -0.5928203230275542746 ) ) ;
#80766=ADVANCED_FACE ( 'NONE', ( #106146 ), #66057, .T. ) ;
#80767=DIRECTION ( 'NONE',  ( 0.000000000000000000, 0.000000000000000000, -1.000000000000000000 ) ) ;
#80768=EDGE_LOOP ( 'NONE', ( #34359, #9867, #104490, #60666 ) ) ;
#80769=AXIS2_PLACEMENT_3D ( 'NONE', #123385, #103757, #82180 ) ;
#80770=DIRECTION ( 'NONE',  ( -0.000000000000000000, 1.000000000000000000, -0.000000000000000000 ) ) ;
#80771=EDGE_CURVE ( 'NONE', #66014, #27399, #76536, .T. ) ;
#80772=EDGE_CURVE ( 'NONE', #53677, #125527, #80563, .T. ) ;
#80773=AXIS2_PLACEMENT_3D ( 'NONE', #117686, #37236, #56830 ) ;
#80774=ADVANCED_FACE ( 'NONE', ( #60296 ), #39367, .T. ) ;
#80775=CIRCLE ( 'NONE', #24323, 0.1000000000000002554 ) ;
#80776=ADVANCED_FACE ( 'NONE', ( #129037 ), #114188, .T. ) ;
#80777=VERTEX_POINT ( 'NONE', #100198 ) ;
#80778=CONICAL_SURFACE ( 'NONE', #112161, 0.1000000000000002554, 0.003490658503988666988 ) ;
#80779=CARTESIAN_POINT ( 'NONE',  ( -9.600000000000006750, 2.500000000000000000, 0.7928203230275495672 ) ) ;
#80780=DIRECTION ( 'NONE',  ( 0.000000000000000000, 0.000000000000000000, 1.000000000000000000 ) ) ;
#80781=AXIS2_PLACEMENT_3D ( 'NONE', #75185, #26099, #5775 ) ;
#80782=EDGE_CURVE ( 'NONE', #53598, #115977, #19033, .T. ) ;
#80785=PLANE ( 'NONE',  #109156 ) ;
#80786=CARTESIAN_POINT ( 'NONE',  ( -13.94999999999998685, 2.500000000000000000, 1.818653347947325472 ) ) ;
#80787=FACE_OUTER_BOUND ( 'NONE', #11312, .T. ) ;
#80788=EDGE_LOOP ( 'NONE', ( #64155, #54567, #85894, #127516 ) ) ;
#80789=EDGE_CURVE ( 'NONE', #82278, #49764, #107827, .T. ) ;
#80790=AXIS2_PLACEMENT_3D ( 'NONE', #93519, #92213, #21555 ) ;
#80791=DIRECTION ( 'NONE',  ( 0.000000000000000000, 1.000000000000000000, 0.000000000000000000 ) ) ;
#80792=AXIS2_PLACEMENT_3D ( 'NONE', #115122, #25464, #105339 ) ;
#80793=AXIS2_PLACEMENT_3D ( 'NONE', #85822, #35461, #117193 ) ;
#80795=CARTESIAN_POINT ( 'NONE',  ( -11.84999999999999609, 12.50000000000000000, 6.841600689897072485 ) ) ;
#80796=EDGE_LOOP ( 'NONE', ( #89681, #19259 ) ) ;
#80797=DIRECTION ( 'NONE',  ( 0.000000000000000000, 0.000000000000000000, 1.000000000000000000 ) ) ;
#80798=ORIENTED_EDGE ( 'NONE', *, *, #15547, .T. ) ;
#80799=ORIENTED_EDGE ( 'NONE', *, *, #5238, .T. ) ;
#80800=DIRECTION ( 'NONE',  ( 0.000000000000000000, 0.000000000000000000, -1.000000000000000000 ) ) ;
#80801=ORIENTED_EDGE ( 'NONE', *, *, #94895, .F. ) ;
#80802=CARTESIAN_POINT ( 'NONE',  ( 17.34645602449680979, -0.4686430837605670696, -5.377443133682146659 ) ) ;
#80803=DIRECTION ( 'NONE',  ( -0.000000000000000000, -1.000000000000000000, -0.000000000000000000 ) ) ;
#80804=LINE ( 'NONE', #120715, #15070 ) ;
#80805=ORIENTED_EDGE ( 'NONE', *, *, #55309, .T. ) ;
#80806=DIRECTION ( 'NONE',  ( 0.000000000000000000, 0.000000000000000000, 1.000000000000000000 ) ) ;
#80807=LINE ( 'NONE', #73537, #93463 ) ;
#80808=FACE_OUTER_BOUND ( 'NONE', #7173, .T. ) ;
#80809=ORIENTED_EDGE ( 'NONE', *, *, #13179, .F. ) ;
#80810=AXIS2_PLACEMENT_3D ( 'NONE', #30815, #91641, #81810 ) ;
#80811=EDGE_CURVE ( 'NONE', #59946, #65442, #79280, .T. ) ;
#80812=ORIENTED_EDGE ( 'NONE', *, *, #55045, .F. ) ;
#80813=CIRCLE ( 'NONE', #78771, 0.09999999999999982514 ) ;
#80814=ORIENTED_EDGE ( 'NONE', *, *, #23932, .F. ) ;
#80815=DIRECTION ( 'NONE',  ( 0.000000000000000000, 1.000000000000000000, 0.000000000000000000 ) ) ;
#80816=CARTESIAN_POINT ( 'NONE',  ( 1.649999999999951505, 12.50000000000000000, 2.857883832488649301 ) ) ;
#80817=CARTESIAN_POINT ( 'NONE',  ( -0.6000000000000383915, 2.500000000000000000, -4.083716857408426826 ) ) ;
#80818=FACE_BOUND ( 'NONE', #52177, .T. ) ;
#80819=EDGE_LOOP ( 'NONE', ( #125721, #22857, #82020, #114047 ) ) ;
#80820=DIRECTION ( 'NONE',  ( 0.000000000000000000, 1.000000000000000000, 0.000000000000000000 ) ) ;
#80821=DIRECTION ( 'NONE',  ( 0.000000000000000000, 0.000000000000000000, -1.000000000000000000 ) ) ;
#80822=EDGE_LOOP ( 'NONE', ( #76189, #120503, #2200, #49705 ) ) ;
#80823=CIRCLE ( 'NONE', #26443, 0.06509327318403743123 ) ;
#80824=VECTOR ( 'NONE', #73716, 1000.000000000000000 ) ;
#80825=ADVANCED_FACE ( 'NONE', ( #91020 ), #119190, .T. ) ;
#80826=CARTESIAN_POINT ( 'NONE',  ( 5.199999999999937117, 2.500000000000000000, -4.576537180435978236 ) ) ;
#80827=DIRECTION ( 'NONE',  ( 0.000000000000000000, 1.000000000000000000, 0.000000000000000000 ) ) ;
#80828=CARTESIAN_POINT ( 'NONE',  ( 3.099999999999944134, 12.50000000000000000, 4.611443907251934426 ) ) ;
#80829=DIRECTION ( 'NONE',  ( 0.000000000000000000, 0.000000000000000000, 1.000000000000000000 ) ) ;
#80830=DIRECTION ( 'NONE',  ( 0.000000000000000000, 1.000000000000000000, 0.000000000000000000 ) ) ;
#80831=CARTESIAN_POINT ( 'NONE',  ( 11.64999999999990798, 12.50000000000000000, 5.802370205355744659 ) ) ;
#80832=DIRECTION ( 'NONE',  ( 0.000000000000000000, -0.9999939076577903929, 0.003490651415223739937 ) ) ;
#80833=AXIS2_PLACEMENT_3D ( 'NONE', #40698, #120525, #70773 ) ;
#80834=AXIS2_PLACEMENT_3D ( 'NONE', #21726, #22384, #72755 ) ;
#80835=CONICAL_SURFACE ( 'NONE', #99617, 0.1000000000000002554, 0.003490658503988666988 ) ;
#80836=VERTEX_POINT ( 'NONE', #51743 ) ;
#80837=EDGE_LOOP ( 'NONE', ( #78446, #123944 ) ) ;
#80838=ORIENTED_EDGE ( 'NONE', *, *, #75507, .F. ) ;
#80839=ORIENTED_EDGE ( 'NONE', *, *, #55756, .F. ) ;
#80840=CARTESIAN_POINT ( 'NONE',  ( -4.119968255444916849E-14, 2.500000000000000000, 3.737306695894644371 ) ) ;
#80841=CARTESIAN_POINT ( 'NONE',  ( 1.849999999999950573, 2.500000000000000000, -1.718653347947326049 ) ) ;
#80842=ORIENTED_EDGE ( 'NONE', *, *, #16341, .F. ) ;
#80843=FACE_BOUND ( 'NONE', #46351, .T. ) ;
#80844=DIRECTION ( 'NONE',  ( -0.000000000000000000, 1.000000000000000000, -0.000000000000000000 ) ) ;
#80845=LINE ( 'NONE', #67263, #99336 ) ;
#80846=DIRECTION ( 'NONE',  ( 0.000000000000000000, 0.000000000000000000, -1.000000000000000000 ) ) ;
#80847=CARTESIAN_POINT ( 'NONE',  ( 5.799999999999931433, 12.50000000000000000, 4.265033745738159077 ) ) ;
#80848=CARTESIAN_POINT ( 'NONE',  ( 4.399999999999937295, 2.500000000000000000, 3.983716857408420964 ) ) ;
#80849=CARTESIAN_POINT ( 'NONE',  ( -10.40000000000000213, 2.500000000000000000, 0.6928203230275494784 ) ) ;
#80850=CARTESIAN_POINT ( 'NONE',  ( -6.850000000000013856, 2.500000000000000000, 6.148780366869520897 ) ) ;
#80851=DIRECTION ( 'NONE',  ( 0.000000000000000000, -0.9999939076577903929, 0.003490651415223739937 ) ) ;
#80852=CIRCLE ( 'NONE', #45352, 0.1000000000000000056 ) ;
#80853=EDGE_LOOP ( 'NONE', ( #80439, #105472, #29543, #73069 ) ) ;
#80854=AXIS2_PLACEMENT_3D ( 'NONE', #77463, #38192, #28376 ) ;
#80855=EDGE_LOOP ( 'NONE', ( #58067, #15281, #7814, #117340 ) ) ;
#80856=EDGE_CURVE ( 'NONE', #25999, #102068, #80748, .T. ) ;
#80857=VERTEX_POINT ( 'NONE', #120478 ) ;
#80858=AXIS2_PLACEMENT_3D ( 'NONE', #35088, #14751, #114903 ) ;
#80859=EDGE_LOOP ( 'NONE', ( #70849, #1810 ) ) ;
#80860=ORIENTED_EDGE ( 'NONE', *, *, #24749, .T. ) ;
#80861=ORIENTED_EDGE ( 'NONE', *, *, #41474, .F. ) ;
#80862=DIRECTION ( 'NONE',  ( -0.000000000000000000, -1.000000000000000000, -0.000000000000000000 ) ) ;
#80863=ORIENTED_EDGE ( 'NONE', *, *, #112943, .F. ) ;
#80864=VECTOR ( 'NONE', #118984, 1000.000000000000000 ) ;
#80865=ADVANCED_FACE ( 'NONE', ( #119829 ), #41047, .T. ) ;
#80866=CIRCLE ( 'NONE', #57884, 0.1000000000000002554 ) ;
#80867=CARTESIAN_POINT ( 'NONE',  ( 19.09982477502542153, 0.5559300837585670063, 4.454172625795878027 ) ) ;
#80869=DIRECTION ( 'NONE',  ( 0.000000000000000000, 1.000000000000000000, 0.000000000000000000 ) ) ;
#80870=DIRECTION ( 'NONE',  ( -0.000000000000000000, -1.000000000000000000, -0.000000000000000000 ) ) ;
#80871=EDGE_CURVE ( 'NONE', #53276, #117920, #91201, .T. ) ;
#80872=AXIS2_PLACEMENT_3D ( 'NONE', #128375, #38715, #78628 ) ;
#80873=EDGE_CURVE ( 'NONE', #122009, #123754, #60905, .T. ) ;
#80874=VERTEX_POINT ( 'NONE', #100817 ) ;
#80876=VECTOR ( 'NONE', #111714, 1000.000000000000000 ) ;
#80878=AXIS2_PLACEMENT_3D ( 'NONE', #27909, #59981, #58028 ) ;
#80879=CIRCLE ( 'NONE', #97585, 0.1000000000000002554 ) ;
#80880=ORIENTED_EDGE ( 'NONE', *, *, #92235, .F. ) ;
#80881=DIRECTION ( 'NONE',  ( 0.000000000000000000, -0.000000000000000000, 1.000000000000000000 ) ) ;
#80882=ADVANCED_FACE ( 'NONE', ( #31461 ), #112038, .T. ) ;
#80883=DIRECTION ( 'NONE',  ( 0.000000000000000000, 0.000000000000000000, 1.000000000000000000 ) ) ;
#80884=CARTESIAN_POINT ( 'NONE',  ( -3.550000000000030909, 2.500000000000000000, -6.841600689897078702 ) ) ;
#80885=ADVANCED_FACE ( 'NONE', ( #38728 ), #7649, .T. ) ;
#80887=VERTEX_POINT ( 'NONE', #98897 ) ;
#80888=FACE_OUTER_BOUND ( 'NONE', #15686, .T. ) ;
#80889=DIRECTION ( 'NONE',  ( 0.000000000000000000, 1.000000000000000000, 0.000000000000000000 ) ) ;
#80890=DIRECTION ( 'NONE',  ( 0.000000000000000000, 0.000000000000000000, 1.000000000000000000 ) ) ;
#80891=PLANE ( 'NONE',  #23177 ) ;
#80892=VERTEX_POINT ( 'NONE', #11804 ) ;
#80893=DIRECTION ( 'NONE',  ( 0.000000000000000000, 1.000000000000000000, 0.000000000000000000 ) ) ;
#80894=CIRCLE ( 'NONE', #18176, 0.06509327318403745899 ) ;
#80895=ORIENTED_EDGE ( 'NONE', *, *, #66068, .T. ) ;
#80896=CARTESIAN_POINT ( 'NONE',  ( 12.31005523242778210, -2.500000000000000000, 7.488833079370801116 ) ) ;
#80897=EDGE_LOOP ( 'NONE', ( #77468, #91275, #69978, #27575 ) ) ;
#80898=DIRECTION ( 'NONE',  ( 0.000000000000000000, 1.000000000000000000, 0.000000000000000000 ) ) ;
#80899=CARTESIAN_POINT ( 'NONE',  ( -5.600000000000020073, 12.50000000000000000, 0.3464101615137736845 ) ) ;
#80900=DIRECTION ( 'NONE',  ( 0.000000000000000000, 1.000000000000000000, 0.000000000000000000 ) ) ;
#80902=ORIENTED_EDGE ( 'NONE', *, *, #121985, .T. ) ;
#80903=DIRECTION ( 'NONE',  ( 0.000000000000000000, 1.000000000000000000, 0.000000000000000000 ) ) ;
#80904=AXIS2_PLACEMENT_3D ( 'NONE', #20171, #60119, #100027 ) ;
#80905=FACE_OUTER_BOUND ( 'NONE', #6228, .T. ) ;
#80906=ORIENTED_EDGE ( 'NONE', *, *, #86209, .F. ) ;
#80907=ORIENTED_EDGE ( 'NONE', *, *, #81198, .F. ) ;
#80908=ORIENTED_EDGE ( 'NONE', *, *, #108092, .F. ) ;
#80909=CARTESIAN_POINT ( 'NONE',  ( 17.50000000000000000, 2.750000000000000000, 4.000000000000001776 ) ) ;
#80910=DIRECTION ( 'NONE',  ( -0.000000000000000000, 1.000000000000000000, -0.000000000000000000 ) ) ;
#80911=CARTESIAN_POINT ( 'NONE',  ( -1.250000000000001554, 2.500000000000000000, 2.165063509461097713 ) ) ;
#80912=DIRECTION ( 'NONE',  ( -0.000000000000000000, -1.000000000000000000, -0.000000000000000000 ) ) ;
#80913=DIRECTION ( 'NONE',  ( 0.000000000000000000, 0.000000000000000000, 1.000000000000000000 ) ) ;
#80914=AXIS2_PLACEMENT_3D ( 'NONE', #5890, #106684, #16979 ) ;
#80915=DIRECTION ( 'NONE',  ( 0.000000000000000000, 1.000000000000000000, 0.000000000000000000 ) ) ;
#80916=AXIS2_PLACEMENT_3D ( 'NONE', #50338, #117761, #9767 ) ;
#80917=ADVANCED_FACE ( 'NONE', ( #89090 ), #112138, .T. ) ;
#80918=CARTESIAN_POINT ( 'NONE',  ( 5.199999999999937117, 2.500000000000000000, -4.576537180435978236 ) ) ;
#80919=CARTESIAN_POINT ( 'NONE',  ( -3.950000000000026379, 2.500000000000000000, 2.511473670974873507 ) ) ;
#80920=LINE ( 'NONE', #59362, #90249 ) ;
#80921=EDGE_CURVE ( 'NONE', #59130, #102506, #34882, .T. ) ;
#80922=EDGE_CURVE ( 'NONE', #74443, #19888, #103813, .T. ) ;
#80923=EDGE_CURVE ( 'NONE', #95802, #87020, #121755, .T. ) ;
#80924=AXIS2_PLACEMENT_3D ( 'NONE', #97335, #125026, #79629 ) ;
#80925=CONICAL_SURFACE ( 'NONE', #34879, 0.09999999999999999167, 0.003490658503988666988 ) ;
#80926=EDGE_CURVE ( 'NONE', #51891, #251, #61959, .T. ) ;
#80927=CONICAL_SURFACE ( 'NONE', #24481, 0.1000000000000002554, 0.003490658503988666988 ) ;
#80928=ORIENTED_EDGE ( 'NONE', *, *, #48427, .T. ) ;
#80929=ADVANCED_FACE ( 'NONE', ( #13075 ), #93347, .T. ) ;
#80930=CARTESIAN_POINT ( 'NONE',  ( -14.59999999999998366, 12.50000000000000000, 0.7579135962115892688 ) ) ;
#80931=DIRECTION ( 'NONE',  ( 0.000000000000000000, 0.000000000000000000, -1.000000000000000000 ) ) ;
#80932=DIRECTION ( 'NONE',  ( -0.000000000000000000, -1.000000000000000000, -0.000000000000000000 ) ) ;
#80933=CARTESIAN_POINT ( 'NONE',  ( 12.29999999999990656, 2.500000000000000000, 3.983716857408420964 ) ) ;
#80934=ORIENTED_EDGE ( 'NONE', *, *, #113089, .F. ) ;
#80935=EDGE_CURVE ( 'NONE', #76431, #18475, #74560, .T. ) ;
#80936=CARTESIAN_POINT ( 'NONE',  ( 4.599999999999937472, 12.50000000000000000, 0.6928203230275494784 ) ) ;
#80937=ADVANCED_FACE ( 'NONE', ( #24214 ), #76624, .T. ) ;
#80938=CARTESIAN_POINT ( 'NONE',  ( 0.7999999999999612976, 2.500000000000000000, -1.084202172485504434E-16 ) ) ;
#80939=CARTESIAN_POINT ( 'NONE',  ( 10.59999999999990905, 12.50000000000000000, -4.611443907251940644 ) ) ;
#80940=ORIENTED_EDGE ( 'NONE', *, *, #125424, .T. ) ;
#80941=CONICAL_SURFACE ( 'NONE', #66258, 0.09999999999999982514, 0.003490658503988666988 ) ;
#80942=ORIENTED_EDGE ( 'NONE', *, *, #58402, .F. ) ;
#80943=AXIS2_PLACEMENT_3D ( 'NONE', #62350, #102269, #83277 ) ;
#80944=DIRECTION ( 'NONE',  ( 0.000000000000000000, -0.000000000000000000, 1.000000000000000000 ) ) ;
#80945=AXIS2_PLACEMENT_3D ( 'NONE', #123928, #6080, #34936 ) ;
#80946=ORIENTED_EDGE ( 'NONE', *, *, #59790, .F. ) ;
#80947=ORIENTED_EDGE ( 'NONE', *, *, #54703, .T. ) ;
#80948=CARTESIAN_POINT ( 'NONE',  ( 9.549999999999918998, 12.50000000000000000, 2.230156782645134950 ) ) ;
#80949=CONICAL_SURFACE ( 'NONE', #16165, 0.09999999999999982514, 0.003490658503988666988 ) ;
#80950=CARTESIAN_POINT ( 'NONE',  ( -6.450000000000016165, 2.500000000000000000, 2.411473670974873862 ) ) ;
#80951=CARTESIAN_POINT ( 'NONE',  ( -13.94999999999998863, 2.500000000000000000, -1.818653347947323917 ) ) ;
#80952=AXIS2_PLACEMENT_3D ( 'NONE', #7573, #84855, #96590 ) ;
#80953=CARTESIAN_POINT ( 'NONE',  ( -1.850000000000033396, 12.50000000000000000, -6.083687093685488989 ) ) ;
#80954=EDGE_LOOP ( 'NONE', ( #84605, #79176, #50967, #84896 ) ) ;
#80955=AXIS2_PLACEMENT_3D ( 'NONE', #28792, #18306, #96212 ) ;
#80956=EDGE_LOOP ( 'NONE', ( #49635, #95773, #43916, #101938 ) ) ;
#80957=CARTESIAN_POINT ( 'NONE',  ( -2.700000000000030820, 2.500000000000000000, 0.3464101615137735735 ) ) ;
#80958=AXIS2_PLACEMENT_3D ( 'NONE', #82976, #82330, #122257 ) ;
#80959=DIRECTION ( 'NONE',  ( 0.000000000000000000, 0.000000000000000000, -1.000000000000000000 ) ) ;
#80960=ORIENTED_EDGE ( 'NONE', *, *, #17474, .F. ) ;
#80961=CIRCLE ( 'NONE', #41266, 0.09999999999999982514 ) ;
#80962=VECTOR ( 'NONE', #122871, 1000.000000000000000 ) ;
#80963=ORIENTED_EDGE ( 'NONE', *, *, #16702, .T. ) ;
#80964=ORIENTED_EDGE ( 'NONE', *, *, #75133, .T. ) ;
#80965=ORIENTED_EDGE ( 'NONE', *, *, #59636, .T. ) ;
#80966=CARTESIAN_POINT ( 'NONE',  ( -7.499999999999980460, 2.500000000000000000, -2.276824562219559311E-15 ) ) ;
#80967=CARTESIAN_POINT ( 'NONE',  ( 8.512291507236481536, 2.500000000000128786, 9.502944100472571876 ) ) ;
#80968=PLANE ( 'NONE',  #92193 ) ;
#80969=FACE_BOUND ( 'NONE', #10592, .T. ) ;
#80970=CARTESIAN_POINT ( 'NONE',  ( 10.39999999999991331, 2.500000000000000000, 0.09999999999999761857 ) ) ;
#80972=FACE_OUTER_BOUND ( 'NONE', #53203, .T. ) ;
#80973=LINE ( 'NONE', #109787, #119066 ) ;
#80974=ADVANCED_FACE ( 'NONE', ( #53031 ), #102128, .T. ) ;
#80975=CARTESIAN_POINT ( 'NONE',  ( -2.300000000000033573, 12.50000000000000000, -3.983716857408426293 ) ) ;
#80976=DIRECTION ( 'NONE',  ( -0.000000000000000000, 1.000000000000000000, -0.000000000000000000 ) ) ;
#80977=AXIS2_PLACEMENT_3D ( 'NONE', #107519, #108789, #7369 ) ;
#80978=DIRECTION ( 'NONE',  ( 0.000000000000000000, 0.000000000000000000, 1.000000000000000000 ) ) ;
#80979=CARTESIAN_POINT ( 'NONE',  ( 12.04999999999990834, 2.500000000000000000, -2.165063509461101710 ) ) ;
#80980=EDGE_LOOP ( 'NONE', ( #101789, #57926 ) ) ;
#80981=ORIENTED_EDGE ( 'NONE', *, *, #53530, .F. ) ;
#80982=VERTEX_POINT ( 'NONE', #103419 ) ;
#80983=ORIENTED_EDGE ( 'NONE', *, *, #47093, .T. ) ;
#80984=EDGE_LOOP ( 'NONE', ( #61228, #119171 ) ) ;
#80985=DIRECTION ( 'NONE',  ( 0.000000000000000000, 0.000000000000000000, -1.000000000000000000 ) ) ;
#80986=DIRECTION ( 'NONE',  ( 0.000000000000000000, 0.000000000000000000, 1.000000000000000000 ) ) ;
#80987=ORIENTED_EDGE ( 'NONE', *, *, #69851, .F. ) ;
#80988=FACE_BOUND ( 'NONE', #115279, .T. ) ;
#80989=DIRECTION ( 'NONE',  ( 0.000000000000000000, -0.000000000000000000, 1.000000000000000000 ) ) ;
#80990=CIRCLE ( 'NONE', #112389, 0.06509327318403745899 ) ;
#80991=VECTOR ( 'NONE', #97034, 1000.000000000000000 ) ;
#80992=ORIENTED_EDGE ( 'NONE', *, *, #30980, .T. ) ;
#80993=FACE_OUTER_BOUND ( 'NONE', #6608, .T. ) ;
#80994=LINE ( 'NONE', #111741, #7589 ) ;
#80995=DIRECTION ( 'NONE',  ( 0.000000000000000000, -0.9999939076577903929, 0.003490651415223739937 ) ) ;
#80996=CARTESIAN_POINT ( 'NONE',  ( 7.499999999999961808, 2.500000000000000000, -4.330127018922201643 ) ) ;
#80997=ORIENTED_EDGE ( 'NONE', *, *, #118585, .F. ) ;
#80998=LINE ( 'NONE', #71170, #103591 ) ;
#80999=AXIS2_PLACEMENT_3D ( 'NONE', #18151, #69844, #109769 ) ;
#81000=AXIS2_PLACEMENT_3D ( 'NONE', #34584, #74487, #65291 ) ;
#81001=AXIS2_PLACEMENT_3D ( 'NONE', #70894, #2790, #100359 ) ;
#81002=ORIENTED_EDGE ( 'NONE', *, *, #54265, .T. ) ;
#81003=VERTEX_POINT ( 'NONE', #13728 ) ;
#81004=CARTESIAN_POINT ( 'NONE',  ( 2.699999999999944666, 2.500000000000000000, 4.676537180435972552 ) ) ;
#81005=DIRECTION ( 'NONE',  ( 0.000000000000000000, 1.000000000000000000, 0.000000000000000000 ) ) ;
#81006=VERTEX_POINT ( 'NONE', #92294 ) ;
#81007=DIRECTION ( 'NONE',  ( 0.000000000000000000, 0.000000000000000000, 1.000000000000000000 ) ) ;
#81008=CONICAL_SURFACE ( 'NONE', #64087, 0.1000000000000000472, 0.003490658503988666988 ) ;
#81009=AXIS2_PLACEMENT_3D ( 'NONE', #21099, #52491, #9998 ) ;
#81010=EDGE_CURVE ( 'NONE', #115678, #13172, #114509, .T. ) ;
#81011=CARTESIAN_POINT ( 'NONE',  ( 7.099999999999928590, 2.500000000000000000, 4.330127018922196314 ) ) ;
#81012=CARTESIAN_POINT ( 'NONE',  ( -12.29999999999999716, 12.50000000000000000, -3.983716857408423628 ) ) ;
#81013=CARTESIAN_POINT ( 'NONE',  ( -9.400000000000007461, 12.50000000000000000, 4.676537180435972552 ) ) ;
#81014=ORIENTED_EDGE ( 'NONE', *, *, #73987, .F. ) ;
#81015=ADVANCED_FACE ( 'NONE', ( #82500 ), #122421, .T. ) ;
#81016=CARTESIAN_POINT ( 'NONE',  ( 12.49999999999990408, 2.500000000000000000, 5.022947341949748790 ) ) ;
#81017=ADVANCED_FACE ( 'NONE', ( #44487 ), #18118, .T. ) ;
#81018=VERTEX_POINT ( 'NONE', #3918 ) ;
#81019=DIRECTION ( 'NONE',  ( 0.000000000000000000, 1.000000000000000000, 0.000000000000000000 ) ) ;
#81020=VECTOR ( 'NONE', #11885, 1000.000000000000000 ) ;
#81021=ORIENTED_EDGE ( 'NONE', *, *, #11035, .T. ) ;
#81022=CARTESIAN_POINT ( 'NONE',  ( -4.200000000000029488, 12.50000000000000000, -4.265033745738164406 ) ) ;
#81023=ORIENTED_EDGE ( 'NONE', *, *, #111947, .F. ) ;
#81024=CARTESIAN_POINT ( 'NONE',  ( -7.900000000000011013, 2.500000000000000000, 4.330127018922196314 ) ) ;
#81025=CIRCLE ( 'NONE', #49737, 0.06509327318403745899 ) ;
#81026=DIRECTION ( 'NONE',  ( 0.000000000000000000, 1.000000000000000000, 0.000000000000000000 ) ) ;
#81027=ADVANCED_FACE ( 'NONE', ( #81826 ), #43869, .T. ) ;
#81028=EDGE_CURVE ( 'NONE', #58821, #94262, #11767, .T. ) ;
#81029=DIRECTION ( 'NONE',  ( 0.000000000000000000, 1.000000000000000000, 0.000000000000000000 ) ) ;
#81030=EDGE_CURVE ( 'NONE', #42019, #87160, #28509, .T. ) ;
#81031=CARTESIAN_POINT ( 'NONE',  ( 10.39999999999991331, 12.50000000000000000, -2.385244779468109755E-15 ) ) ;
#81032=EDGE_CURVE ( 'NONE', #67345, #49421, #34031, .T. ) ;
#81033=EDGE_CURVE ( 'NONE', #127662, #66202, #104059, .T. ) ;
#81034=CARTESIAN_POINT ( 'NONE',  ( -7.499999999999976907, 2.500000000000000000, 4.330127018922196314 ) ) ;
#81035=AXIS2_PLACEMENT_3D ( 'NONE', #96142, #45125, #74575 ) ;
#81036=VERTEX_POINT ( 'NONE', #72672 ) ;
#81037=AXIS2_PLACEMENT_3D ( 'NONE', #39973, #79886, #70073 ) ;
#81038=ORIENTED_EDGE ( 'NONE', *, *, #32070, .F. ) ;
#81039=EDGE_LOOP ( 'NONE', ( #84751, #12909 ) ) ;
#81041=AXIS2_PLACEMENT_3D ( 'NONE', #108926, #8156, #77541 ) ;
#81043=DIRECTION ( 'NONE',  ( 0.000000000000000000, 1.000000000000000000, 0.000000000000000000 ) ) ;
#81044=VERTEX_POINT ( 'NONE', #104685 ) ;
#81045=VERTEX_POINT ( 'NONE', #23561 ) ;
#81046=VERTEX_POINT ( 'NONE', #32115 ) ;
#81047=ADVANCED_FACE ( 'NONE', ( #72033 ), #22300, .T. ) ;
#81048=DIRECTION ( 'NONE',  ( -4.274815082592931898E-19, -0.9999939076577903929, -0.003490651415223739937 ) ) ;
#81049=VECTOR ( 'NONE', #35614, 1000.000000000000000 ) ;
#81050=CIRCLE ( 'NONE', #24602, 0.1000000000000000472 ) ;
#81052=CARTESIAN_POINT ( 'NONE',  ( 10.84999999999990905, 2.500000000000000000, 2.165063509461097713 ) ) ;
#81053=DIRECTION ( 'NONE',  ( 0.000000000000000000, 0.000000000000000000, -1.000000000000000000 ) ) ;
#81054=DIRECTION ( 'NONE',  ( 0.000000000000000000, 1.000000000000000000, 0.000000000000000000 ) ) ;
#81055=DIRECTION ( 'NONE',  ( -1.000000000000000000, -0.000000000000000000, -0.000000000000000000 ) ) ;
#81056=CARTESIAN_POINT ( 'NONE',  ( 11.89999999999990798, 2.500000000000000000, 4.776537180435972196 ) ) ;
#81057=DIRECTION ( 'NONE',  ( 0.000000000000000000, 0.000000000000000000, -1.000000000000000000 ) ) ;
#81058=CARTESIAN_POINT ( 'NONE',  ( 9.599999999999914380, 2.500000000000000000, 4.922947341949748257 ) ) ;
#81059=CONICAL_SURFACE ( 'NONE', #24613, 0.1000000000000000472, 0.003490658503988666988 ) ;
#81060=DIRECTION ( 'NONE',  ( 0.000000000000000000, 0.000000000000000000, 1.000000000000000000 ) ) ;
#81061=EDGE_LOOP ( 'NONE', ( #43000, #15493, #19549, #84011 ) ) ;
#81062=DIRECTION ( 'NONE',  ( -0.000000000000000000, 1.000000000000000000, -0.000000000000000000 ) ) ;
#81063=CONICAL_SURFACE ( 'NONE', #24618, 0.1000000000000002554, 0.003490658503988666988 ) ;
#81064=AXIS2_PLACEMENT_3D ( 'NONE', #107508, #117288, #7358 ) ;
#81065=CARTESIAN_POINT ( 'NONE',  ( -5.650000000000023448, 12.50000000000000000, -6.841600689897078702 ) ) ;
#81066=ORIENTED_EDGE ( 'NONE', *, *, #107016, .T. ) ;
#81067=EDGE_LOOP ( 'NONE', ( #102297, #61491 ) ) ;
#81069=DIRECTION ( 'NONE',  ( 0.000000000000000000, 1.000000000000000000, 0.000000000000000000 ) ) ;
#81070=CARTESIAN_POINT ( 'NONE',  ( -0.4000000000000396572, 2.500000000000000000, 3.737306695894644371 ) ) ;
#81071=CARTESIAN_POINT ( 'NONE',  ( 3.949999999999939782, 2.500000000000000000, 2.411473670974873862 ) ) ;
#81072=LINE ( 'NONE', #72547, #40212 ) ;
#81073=DIRECTION ( 'NONE',  ( 0.000000000000000000, -0.000000000000000000, 1.000000000000000000 ) ) ;
#81074=DIRECTION ( 'NONE',  ( 0.000000000000000000, 1.000000000000000000, 0.000000000000000000 ) ) ;
#81075=DIRECTION ( 'NONE',  ( 0.000000000000000000, -0.9999939076577903929, 0.003490651415223739937 ) ) ;
#81076=EDGE_CURVE ( 'NONE', #54453, #12380, #117080, .T. ) ;
#81077=EDGE_CURVE ( 'NONE', #71302, #108547, #110075, .T. ) ;
#81078=FACE_OUTER_BOUND ( 'NONE', #96833, .T. ) ;
#81079=VERTEX_POINT ( 'NONE', #5195 ) ;
#81081=EDGE_CURVE ( 'NONE', #22283, #5141, #124735, .T. ) ;
#81082=EDGE_LOOP ( 'NONE', ( #98260, #27659 ) ) ;
#81083=CIRCLE ( 'NONE', #31025, 0.06509327318403745899 ) ;
#81084=EDGE_LOOP ( 'NONE', ( #14857, #105047 ) ) ;
#81085=ADVANCED_FACE ( 'NONE', ( #46414 ), #80835, .T. ) ;
#81086=ORIENTED_EDGE ( 'NONE', *, *, #50875, .F. ) ;
#81087=DIRECTION ( 'NONE',  ( 0.000000000000000000, 0.000000000000000000, 1.000000000000000000 ) ) ;
#81088=DIRECTION ( 'NONE',  ( 0.000000000000000000, -0.000000000000000000, 1.000000000000000000 ) ) ;
#81089=ADVANCED_FACE ( 'NONE', ( #126930 ), #51500, .T. ) ;
#81090=EDGE_LOOP ( 'NONE', ( #113390, #45006 ) ) ;
#81091=CONICAL_SURFACE ( 'NONE', #79037, 0.1000000000000002554, 0.003490658503988666988 ) ;
#81092=ADVANCED_FACE ( 'NONE', ( #7780 ), #120538, .T. ) ;
#81093=DIRECTION ( 'NONE',  ( 0.000000000000000000, 0.000000000000000000, -1.000000000000000000 ) ) ;
#81094=CONICAL_SURFACE ( 'NONE', #24649, 0.1000000000000002554, 0.003490658503988666988 ) ;
#81095=DIRECTION ( 'NONE',  ( 0.000000000000000000, 0.000000000000000000, 1.000000000000000000 ) ) ;
#81096=ADVANCED_FACE ( 'NONE', ( #125613 ), #96161, .T. ) ;
#81097=DIRECTION ( 'NONE',  ( 0.000000000000000000, 0.000000000000000000, 1.000000000000000000 ) ) ;
#81098=DIRECTION ( 'NONE',  ( 0.000000000000000000, 1.000000000000000000, 0.000000000000000000 ) ) ;
#81099=EDGE_LOOP ( 'NONE', ( #38267, #37709 ) ) ;
#81100=CARTESIAN_POINT ( 'NONE',  ( -1.250000000000001554, 2.500000000000000000, 6.395190528383296602 ) ) ;
#81101=EDGE_CURVE ( 'NONE', #46700, #87285, #78698, .T. ) ;
#81102=VECTOR ( 'NONE', #21651, 1000.000000000000000 ) ;
#81103=CARTESIAN_POINT ( 'NONE',  ( -0.8500000000000386136, 2.500000000000000000, 1.472243186433545459 ) ) ;
#81104=ORIENTED_EDGE ( 'NONE', *, *, #80771, .T. ) ;
#81105=AXIS2_PLACEMENT_3D ( 'NONE', #42585, #20987, #71362 ) ;
#81106=CONICAL_SURFACE ( 'NONE', #118643, 0.1000000000000002554, 0.003490658503988666988 ) ;
#81107=EDGE_LOOP ( 'NONE', ( #63744, #77035 ) ) ;
#81108=ORIENTED_EDGE ( 'NONE', *, *, #110883, .T. ) ;
#81109=ORIENTED_EDGE ( 'NONE', *, *, #106733, .F. ) ;
#81110=FACE_OUTER_BOUND ( 'NONE', #77748, .T. ) ;
#81111=DIRECTION ( 'NONE',  ( 0.000000000000000000, 0.000000000000000000, -1.000000000000000000 ) ) ;
#81112=CARTESIAN_POINT ( 'NONE',  ( -11.44999999999999751, 2.500000000000000000, -6.741600689897073728 ) ) ;
#81113=DIRECTION ( 'NONE',  ( 0.000000000000000000, 1.000000000000000000, 0.000000000000000000 ) ) ;
#81114=ORIENTED_EDGE ( 'NONE', *, *, #18647, .F. ) ;
#81115=CIRCLE ( 'NONE', #41413, 0.06509327318403745899 ) ;
#81116=CARTESIAN_POINT ( 'NONE',  ( -13.54999999999998828, 12.50000000000000000, -2.511473670974875727 ) ) ;
#81117=LINE ( 'NONE', #20897, #66366 ) ;
#81118=DIRECTION ( 'NONE',  ( 0.000000000000000000, 0.000000000000000000, 1.000000000000000000 ) ) ;
#81119=DIRECTION ( 'NONE',  ( 0.000000000000000000, 0.000000000000000000, 1.000000000000000000 ) ) ;
#81120=EDGE_CURVE ( 'NONE', #118657, #28229, #47724, .T. ) ;
#81121=EDGE_LOOP ( 'NONE', ( #92129, #58670 ) ) ;
#81122=AXIS2_PLACEMENT_3D ( 'NONE', #9963, #91742, #2058 ) ;
#81123=CIRCLE ( 'NONE', #87355, 0.1000000000000000472 ) ;
#81124=ORIENTED_EDGE ( 'NONE', *, *, #17805, .T. ) ;
#81125=EDGE_LOOP ( 'NONE', ( #41387, #106866 ) ) ;
#81126=CARTESIAN_POINT ( 'NONE',  ( 5.199999999999931788, 2.500000000000000000, 4.676537180435972552 ) ) ;
#81127=LINE ( 'NONE', #2535, #102489 ) ;
#81128=FACE_BOUND ( 'NONE', #128603, .T. ) ;
#81129=AXIS2_PLACEMENT_3D ( 'NONE', #50594, #90520, #859 ) ;
#81130=DIRECTION ( 'NONE',  ( -0.000000000000000000, 1.000000000000000000, -0.000000000000000000 ) ) ;
#81131=DIRECTION ( 'NONE',  ( 0.000000000000000000, 0.000000000000000000, 1.000000000000000000 ) ) ;
#81132=CIRCLE ( 'NONE', #20490, 0.09999999999999999167 ) ;
#81133=DIRECTION ( 'NONE',  ( -4.274815082592931898E-19, -0.9999939076577903929, -0.003490651415223739937 ) ) ;
#81134=AXIS2_PLACEMENT_3D ( 'NONE', #95754, #114737, #23799 ) ;
#81135=EDGE_CURVE ( 'NONE', #114764, #22907, #118380, .T. ) ;
#81136=CARTESIAN_POINT ( 'NONE',  ( 2.099999999999947686, 2.500000000000000000, 5.122947341949749323 ) ) ;
#81137=CIRCLE ( 'NONE', #5600, 0.1000000000000002554 ) ;
#81138=LINE ( 'NONE', #90276, #117655 ) ;
#81139=CARTESIAN_POINT ( 'NONE',  ( -1.250000000000035749, 12.50000000000000000, -2.792790559304616504 ) ) ;
#81140=EDGE_LOOP ( 'NONE', ( #337, #19979 ) ) ;
#81141=DIRECTION ( 'NONE',  ( -4.274815082592931898E-19, -0.9999939076577903929, -0.003490651415223739937 ) ) ;
#81143=ORIENTED_EDGE ( 'NONE', *, *, #111742, .F. ) ;
#81144=ORIENTED_EDGE ( 'NONE', *, *, #31447, .F. ) ;
#81145=DIRECTION ( 'NONE',  ( 0.000000000000000000, 0.000000000000000000, -1.000000000000000000 ) ) ;
#81146=AXIS2_PLACEMENT_3D ( 'NONE', #23668, #83246, #53135 ) ;
#81147=EDGE_CURVE ( 'NONE', #25877, #42358, #49452, .T. ) ;
#81148=DIRECTION ( 'NONE',  ( 0.000000000000000000, 0.000000000000000000, 1.000000000000000000 ) ) ;
#81149=FACE_BOUND ( 'NONE', #8903, .T. ) ;
#81150=CARTESIAN_POINT ( 'NONE',  ( 13.09999999999990195, 2.500000000000000000, -4.083716857408426826 ) ) ;
#81151=VECTOR ( 'NONE', #24071, 1000.000000000000000 ) ;
#81152=CONICAL_SURFACE ( 'NONE', #16359, 0.09999999999999982514, 0.003490658503988666988 ) ;
#81153=FACE_BOUND ( 'NONE', #115387, .T. ) ;
#81154=EDGE_LOOP ( 'NONE', ( #108240, #73479 ) ) ;
#81155=CARTESIAN_POINT ( 'NONE',  ( 8.749999999999918288, 2.500000000000000000, -1.472243186433550122 ) ) ;
#81157=ORIENTED_EDGE ( 'NONE', *, *, #60426, .F. ) ;
#81158=LINE ( 'NONE', #111228, #11402 ) ;
#81159=DIRECTION ( 'NONE',  ( -0.000000000000000000, 1.000000000000000000, -0.000000000000000000 ) ) ;
#81160=CARTESIAN_POINT ( 'NONE',  ( -10.20000000000000462, 2.500000000000000000, 4.576537180435972019 ) ) ;
#81161=FACE_OUTER_BOUND ( 'NONE', #29531, .T. ) ;
#81162=ORIENTED_EDGE ( 'NONE', *, *, #109271, .T. ) ;
#81163=EDGE_CURVE ( 'NONE', #18723, #88124, #126801, .T. ) ;
#81164=DIRECTION ( 'NONE',  ( 0.000000000000000000, 0.000000000000000000, 1.000000000000000000 ) ) ;
#81165=CARTESIAN_POINT ( 'NONE',  ( 4.999999999999973355, 12.50000000000000000, -4.265033745738164406 ) ) ;
#81166=AXIS2_PLACEMENT_3D ( 'NONE', #54943, #94875, #54308 ) ;
#81167=CARTESIAN_POINT ( 'NONE',  ( 8.749999999999923617, 2.500000000000000000, 1.572243186433545548 ) ) ;
#81168=ORIENTED_EDGE ( 'NONE', *, *, #67621, .F. ) ;
#81169=ORIENTED_EDGE ( 'NONE', *, *, #57511, .F. ) ;
#81170=LINE ( 'NONE', #42554, #24237 ) ;
#81171=ADVANCED_FACE ( 'NONE', ( #77803 ), #114266, .T. ) ;
#81172=EDGE_LOOP ( 'NONE', ( #52548, #107421 ) ) ;
#81173=FACE_OUTER_BOUND ( 'NONE', #9845, .T. ) ;
#81174=CARTESIAN_POINT ( 'NONE',  ( 1.249999999999988454, 2.500000000000000000, -2.165063509461101710 ) ) ;
#81175=AXIS2_PLACEMENT_3D ( 'NONE', #66121, #24269, #125045 ) ;
#81176=DIRECTION ( 'NONE',  ( 0.000000000000000000, 0.000000000000000000, 1.000000000000000000 ) ) ;
#81177=ORIENTED_EDGE ( 'NONE', *, *, #14659, .F. ) ;
#81178=DIRECTION ( 'NONE',  ( 0.000000000000000000, 0.000000000000000000, 1.000000000000000000 ) ) ;
#81179=PLANE ( 'NONE',  #97879 ) ;
#81180=CARTESIAN_POINT ( 'NONE',  ( 9.599999999999914380, 12.50000000000000000, -4.330127018922201643 ) ) ;
#81181=EDGE_CURVE ( 'NONE', #3394, #63089, #17596, .T. ) ;
#81182=ADVANCED_FACE ( 'NONE', ( #116442 ), #99239, .T. ) ;
#81183=CARTESIAN_POINT ( 'NONE',  ( -6.249999999999981348, 2.500000000000000000, 2.065063509461097624 ) ) ;
#81184=DIRECTION ( 'NONE',  ( 0.000000000000000000, 0.000000000000000000, 1.000000000000000000 ) ) ;
#81185=EDGE_CURVE ( 'NONE', #89603, #71314, #103353, .T. ) ;
#81187=DIRECTION ( 'NONE',  ( -0.000000000000000000, -1.000000000000000000, -0.000000000000000000 ) ) ;
#81188=CIRCLE ( 'NONE', #26806, 0.1000000000000002554 ) ;
#81189=EDGE_LOOP ( 'NONE', ( #88093, #44742, #57232, #15927 ) ) ;
#81190=CIRCLE ( 'NONE', #62321, 0.06509327318403741736 ) ;
#81191=ORIENTED_EDGE ( 'NONE', *, *, #78946, .F. ) ;
#81192=DIRECTION ( 'NONE',  ( 0.000000000000000000, 0.000000000000000000, 1.000000000000000000 ) ) ;
#81193=VERTEX_POINT ( 'NONE', #35964 ) ;
#81194=FACE_OUTER_BOUND ( 'NONE', #50025, .T. ) ;
#81196=ORIENTED_EDGE ( 'NONE', *, *, #124698, .T. ) ;
#81197=ORIENTED_EDGE ( 'NONE', *, *, #124203, .F. ) ;
#81198=EDGE_CURVE ( 'NONE', #113969, #91010, #75880, .T. ) ;
#81199=DIRECTION ( 'NONE',  ( 0.000000000000000000, 0.000000000000000000, 1.000000000000000000 ) ) ;
#81200=EDGE_CURVE ( 'NONE', #67150, #48754, #21879, .T. ) ;
#81201=CIRCLE ( 'NONE', #87438, 0.1000000000000002554 ) ;
#81202=PLANE ( 'NONE',  #61125 ) ;
#81203=EDGE_CURVE ( 'NONE', #87409, #105515, #42823, .T. ) ;
#81204=DIRECTION ( 'NONE',  ( 0.000000000000000000, 1.000000000000000000, 0.000000000000000000 ) ) ;
#81206=CARTESIAN_POINT ( 'NONE',  ( 1.649999999999949729, 2.500000000000000000, 7.188010851410848723 ) ) ;
#81207=LINE ( 'NONE', #69432, #96098 ) ;
#81208=DIRECTION ( 'NONE',  ( 0.000000000000000000, 0.000000000000000000, -1.000000000000000000 ) ) ;
#81209=CARTESIAN_POINT ( 'NONE',  ( -5.850000000000022737, 12.50000000000000000, -6.430097255199264339 ) ) ;
#81210=VECTOR ( 'NONE', #66252, 1000.000000000000000 ) ;
#81211=PLANE ( 'NONE',  #59453 ) ;
#81212=CARTESIAN_POINT ( 'NONE',  ( 14.14999999999989377, 12.50000000000000000, -2.857883832488653741 ) ) ;
#81213=CONICAL_SURFACE ( 'NONE', #31055, 0.1000000000000002554, 0.003490658503988666988 ) ;
#81216=CARTESIAN_POINT ( 'NONE',  ( -2.700000000000029932, 12.50000000000000000, -0.3464101615137782364 ) ) ;
#81217=EDGE_LOOP ( 'NONE', ( #11632, #16774, #121334, #25000 ) ) ;
#81218=ORIENTED_EDGE ( 'NONE', *, *, #75394, .T. ) ;
#81219=CARTESIAN_POINT ( 'NONE',  ( 12.49999999999990052, 2.500000000000000000, 0.6928203230275494784 ) ) ;
#81220=CIRCLE ( 'NONE', #129266, 0.1000000000000002554 ) ;
#81221=DIRECTION ( 'NONE',  ( 0.000000000000000000, 1.000000000000000000, 0.000000000000000000 ) ) ;
#81222=DIRECTION ( 'NONE',  ( -0.000000000000000000, -1.000000000000000000, -0.000000000000000000 ) ) ;
#81223=CONICAL_SURFACE ( 'NONE', #112529, 0.1000000000000002554, 0.003490658503988666988 ) ;
#81224=CARTESIAN_POINT ( 'NONE',  ( 11.44999999999990692, 12.50000000000000000, -6.906693963081115939 ) ) ;
#81225=DIRECTION ( 'NONE',  ( 0.000000000000000000, -0.000000000000000000, 1.000000000000000000 ) ) ;
#81226=DIRECTION ( 'NONE',  ( -0.000000000000000000, 1.000000000000000000, -0.000000000000000000 ) ) ;
#81227=ORIENTED_EDGE ( 'NONE', *, *, #108531, .F. ) ;
#81228=AXIS2_PLACEMENT_3D ( 'NONE', #59779, #30953, #29017 ) ;
#81229=ORIENTED_EDGE ( 'NONE', *, *, #42685, .F. ) ;
#81230=ORIENTED_EDGE ( 'NONE', *, *, #73, .T. ) ;
#81231=CARTESIAN_POINT ( 'NONE',  ( 3.149999999999944400, 2.500000000000000000, 2.411473670974873862 ) ) ;
#81232=ORIENTED_EDGE ( 'NONE', *, *, #9825, .T. ) ;
#81233=AXIS2_PLACEMENT_3D ( 'NONE', #63279, #105128, #15448 ) ;
#81234=ADVANCED_FACE ( 'NONE', ( #38567 ), #129529, .T. ) ;
#81235=ORIENTED_EDGE ( 'NONE', *, *, #60668, .F. ) ;
#81236=CARTESIAN_POINT ( 'NONE',  ( 5.599999999999934808, 2.500000000000000000, -4.676537180435978769 ) ) ;
#81237=DIRECTION ( 'NONE',  ( 0.000000000000000000, 0.000000000000000000, 1.000000000000000000 ) ) ;
#81238=ADVANCED_FACE ( 'NONE', ( #60762 ), #69270, .T. ) ;
#81239=AXIS2_PLACEMENT_3D ( 'NONE', #12710, #22577, #62496 ) ;
#81240=AXIS2_PLACEMENT_3D ( 'NONE', #46987, #107824, #116345 ) ;
#81241=CARTESIAN_POINT ( 'NONE',  ( 4.999999999999935163, 2.500000000000000000, 0.7928203230275495672 ) ) ;
#81242=CARTESIAN_POINT ( 'NONE',  ( 2.299999999999949640, 12.50000000000000000, -4.676537180435977881 ) ) ;
#81243=EDGE_CURVE ( 'NONE', #59490, #73228, #17647, .T. ) ;
#81244=CARTESIAN_POINT ( 'NONE',  ( 9.149999999999920419, 2.500000000000000000, -7.188010851410854052 ) ) ;
#81245=EDGE_LOOP ( 'NONE', ( #109801, #98304 ) ) ;
#81246=CARTESIAN_POINT ( 'NONE',  ( 9.149999999999915090, 12.50000000000000000, 6.430097255199259010 ) ) ;
#81247=CARTESIAN_POINT ( 'NONE',  ( 1.049999999999954969, 12.50000000000000000, -6.841600689897077814 ) ) ;
#81248=FACE_OUTER_BOUND ( 'NONE', #89467, .T. ) ;
#81249=FACE_OUTER_BOUND ( 'NONE', #82486, .T. ) ;
#81250=ADVANCED_FACE ( 'NONE', ( #118381 ), #59554, .T. ) ;
#81251=CARTESIAN_POINT ( 'NONE',  ( 4.199999999999938005, 12.50000000000000000, 4.330127018922196314 ) ) ;
#81252=ORIENTED_EDGE ( 'NONE', *, *, #114124, .F. ) ;
#81253=VERTEX_POINT ( 'NONE', #532 ) ;
#81254=VERTEX_POINT ( 'NONE', #68638 ) ;
#81255=FACE_OUTER_BOUND ( 'NONE', #62212, .T. ) ;
#81256=ORIENTED_EDGE ( 'NONE', *, *, #54866, .F. ) ;
#81257=DIRECTION ( 'NONE',  ( 0.000000000000000000, -0.000000000000000000, 1.000000000000000000 ) ) ;
#81258=DIRECTION ( 'NONE',  ( 0.000000000000000000, 0.000000000000000000, 1.000000000000000000 ) ) ;
#81259=AXIS2_PLACEMENT_3D ( 'NONE', #24898, #65455, #126327 ) ;
#81260=CIRCLE ( 'NONE', #49980, 0.09999999999999982514 ) ;
#81261=CIRCLE ( 'NONE', #89574, 0.09999999999999982514 ) ;
#81262=ORIENTED_EDGE ( 'NONE', *, *, #46022, .F. ) ;
#81263=DIRECTION ( 'NONE',  ( -0.000000000000000000, -1.000000000000000000, -0.000000000000000000 ) ) ;
#81264=DIRECTION ( 'NONE',  ( 0.000000000000000000, 0.000000000000000000, -1.000000000000000000 ) ) ;
#81265=DIRECTION ( 'NONE',  ( 0.000000000000000000, 0.000000000000000000, -1.000000000000000000 ) ) ;
#81266=ADVANCED_FACE ( 'NONE', ( #110498 ), #101286, .T. ) ;
#81267=CARTESIAN_POINT ( 'NONE',  ( -1.650000000000035216, 12.50000000000000000, -1.472243186433550122 ) ) ;
#81268=AXIS2_PLACEMENT_3D ( 'NONE', #118843, #88744, #99218 ) ;
#81269=CONICAL_SURFACE ( 'NONE', #33263, 0.1000000000000002554, 0.003490658503988666988 ) ;
#81270=FACE_OUTER_BOUND ( 'NONE', #89110, .T. ) ;
#81271=AXIS2_PLACEMENT_3D ( 'NONE', #27706, #99039, #66976 ) ;
#81272=VERTEX_POINT ( 'NONE', #88258 ) ;
#81273=ORIENTED_EDGE ( 'NONE', *, *, #1867, .T. ) ;
#81274=CARTESIAN_POINT ( 'NONE',  ( -0.4000000000000339950, 2.500000000000000000, 0.5928203230275517210 ) ) ;
#81275=DIRECTION ( 'NONE',  ( -0.000000000000000000, 1.000000000000000000, -0.000000000000000000 ) ) ;
#81276=VECTOR ( 'NONE', #48777, 1000.000000000000000 ) ;
#81277=LINE ( 'NONE', #80638, #120302 ) ;
#81278=DIRECTION ( 'NONE',  ( 0.000000000000000000, 0.000000000000000000, 1.000000000000000000 ) ) ;
#81279=VECTOR ( 'NONE', #98131, 1000.000000000000000 ) ;
#81280=ORIENTED_EDGE ( 'NONE', *, *, #72002, .T. ) ;
#81281=ADVANCED_FACE ( 'NONE', ( #40500 ), #28731, .T. ) ;
#81282=ORIENTED_EDGE ( 'NONE', *, *, #126690, .F. ) ;
#81283=DIRECTION ( 'NONE',  ( 0.000000000000000000, 0.000000000000000000, -1.000000000000000000 ) ) ;
#81284=CARTESIAN_POINT ( 'NONE',  ( -3.750000000000026201, 12.50000000000000000, 5.802370205355744659 ) ) ;
#81285=DIRECTION ( 'NONE',  ( -0.000000000000000000, -1.000000000000000000, -0.000000000000000000 ) ) ;
#81286=VERTEX_POINT ( 'NONE', #109197 ) ;
#81287=CONICAL_SURFACE ( 'NONE', #64548, 0.1000000000000002554, 0.003490658503988666988 ) ;
#81288=LINE ( 'NONE', #120564, #42696 ) ;
#81289=DIRECTION ( 'NONE',  ( 0.000000000000000000, 0.000000000000000000, -1.000000000000000000 ) ) ;
#81290=VECTOR ( 'NONE', #49865, 1000.000000000000000 ) ;
#81291=VERTEX_POINT ( 'NONE', #80410 ) ;
#81292=DIRECTION ( 'NONE',  ( -0.000000000000000000, 1.000000000000000000, -0.000000000000000000 ) ) ;
#81293=EDGE_CURVE ( 'NONE', #30241, #61867, #46918, .T. ) ;
#81294=EDGE_LOOP ( 'NONE', ( #85246, #88480, #69993, #70613 ) ) ;
#81295=LINE ( 'NONE', #121207, #34918 ) ;
#81296=ORIENTED_EDGE ( 'NONE', *, *, #67430, .F. ) ;
#81297=ORIENTED_EDGE ( 'NONE', *, *, #74021, .F. ) ;
#81299=CARTESIAN_POINT ( 'NONE',  ( 1.899999999999949507, 2.500000000000000000, 4.576537180435972019 ) ) ;
#81300=CARTESIAN_POINT ( 'NONE',  ( 14.69205215198098102, 2.499999999999999556, -6.336420067969235959 ) ) ;
#81301=ORIENTED_EDGE ( 'NONE', *, *, #46398, .F. ) ;
#81302=EDGE_CURVE ( 'NONE', #36694, #124473, #34410, .T. ) ;
#81303=EDGE_LOOP ( 'NONE', ( #116937, #84889, #55763, #129032 ) ) ;
#81304=DIRECTION ( 'NONE',  ( 0.000000000000000000, 0.000000000000000000, -1.000000000000000000 ) ) ;
#81305=DIRECTION ( 'NONE',  ( 0.000000000000000000, 0.000000000000000000, -1.000000000000000000 ) ) ;
#81306=AXIS2_PLACEMENT_3D ( 'NONE', #122736, #33093, #114207 ) ;
#81307=ORIENTED_EDGE ( 'NONE', *, *, #89940, .T. ) ;
#81310=AXIS2_PLACEMENT_3D ( 'NONE', #93349, #92704, #3041 ) ;
#81311=FACE_OUTER_BOUND ( 'NONE', #107541, .T. ) ;
#81312=DIRECTION ( 'NONE',  ( 0.000000000000000000, 0.000000000000000000, 1.000000000000000000 ) ) ;
#81313=CARTESIAN_POINT ( 'NONE',  ( 7.899999999999924860, 12.50000000000000000, 4.957854068765711553 ) ) ;
#81314=DIRECTION ( 'NONE',  ( -0.000000000000000000, 1.000000000000000000, -0.000000000000000000 ) ) ;
#81317=VERTEX_POINT ( 'NONE', #128223 ) ;
#81318=ADVANCED_FACE ( 'NONE', ( #90860 ), #100663, .T. ) ;
#81319=ORIENTED_EDGE ( 'NONE', *, *, #6247, .T. ) ;
#81320=CARTESIAN_POINT ( 'NONE',  ( -12.69999999999999041, 2.500000000000000000, 4.083716857408421497 ) ) ;
#81321=AXIS2_PLACEMENT_3D ( 'NONE', #41337, #100244, #21026 ) ;
#81322=AXIS2_PLACEMENT_3D ( 'NONE', #72602, #5757, #103351 ) ;
#81323=ORIENTED_EDGE ( 'NONE', *, *, #113241, .T. ) ;
#81324=FACE_OUTER_BOUND ( 'NONE', #78370, .T. ) ;
#81325=CARTESIAN_POINT ( 'NONE',  ( -5.450000000000019718, 2.500000000000000000, 6.395190528383296602 ) ) ;
#81326=PLANE ( 'NONE',  #34381 ) ;
#81327=ORIENTED_EDGE ( 'NONE', *, *, #72882, .T. ) ;
#81328=ORIENTED_EDGE ( 'NONE', *, *, #82783, .T. ) ;
#81329=FACE_BOUND ( 'NONE', #90148, .T. ) ;
#81330=ORIENTED_EDGE ( 'NONE', *, *, #83711, .T. ) ;
#81331=CARTESIAN_POINT ( 'NONE',  ( 6.049999999999930544, 2.500000000000000000, 2.511473670974873507 ) ) ;
#81332=DIRECTION ( 'NONE',  ( 0.000000000000000000, 0.000000000000000000, -1.000000000000000000 ) ) ;
#81333=DIRECTION ( 'NONE',  ( -0.000000000000000000, 1.000000000000000000, -0.000000000000000000 ) ) ;
#81334=ADVANCED_FACE ( 'NONE', ( #59503 ), #7180, .T. ) ;
#81335=CIRCLE ( 'NONE', #6085, 0.1000000000000002554 ) ;
#81336=AXIS2_PLACEMENT_3D ( 'NONE', #82891, #23961, #12817 ) ;
#81337=DIRECTION ( 'NONE',  ( -0.000000000000000000, 1.000000000000000000, -0.000000000000000000 ) ) ;
#81338=DIRECTION ( 'NONE',  ( -0.000000000000000000, -1.000000000000000000, -0.000000000000000000 ) ) ;
#81339=DIRECTION ( 'NONE',  ( 0.000000000000000000, 1.000000000000000000, 0.000000000000000000 ) ) ;
#81340=CARTESIAN_POINT ( 'NONE',  ( 0.5999999999999555689, 12.50000000000000000, 4.741630453620009789 ) ) ;
#81341=DIRECTION ( 'NONE',  ( 0.000000000000000000, 0.000000000000000000, -1.000000000000000000 ) ) ;
#81342=EDGE_CURVE ( 'NONE', #76788, #20030, #1189, .T. ) ;
#81343=EDGE_CURVE ( 'NONE', #120641, #80322, #97077, .T. ) ;
#81344=DIRECTION ( 'NONE',  ( -0.000000000000000000, -1.000000000000000000, -0.000000000000000000 ) ) ;
#81345=DIRECTION ( 'NONE',  ( -0.000000000000000000, 1.000000000000000000, -0.000000000000000000 ) ) ;
#81346=EDGE_CURVE ( 'NONE', #27663, #86126, #44864, .T. ) ;
#81347=EDGE_CURVE ( 'NONE', #47691, #68346, #39216, .T. ) ;
#81348=CARTESIAN_POINT ( 'NONE',  ( 11.44999999999991047, 12.50000000000000000, -2.446380397790840266 ) ) ;
#81349=EDGE_LOOP ( 'NONE', ( #43387, #5323 ) ) ;
#81350=ORIENTED_EDGE ( 'NONE', *, *, #120857, .F. ) ;
#81351=VERTEX_POINT ( 'NONE', #63335 ) ;
#81352=ORIENTED_EDGE ( 'NONE', *, *, #120078, .T. ) ;
#81353=CARTESIAN_POINT ( 'NONE',  ( 2.299999999999949640, 2.500000000000000000, -4.576537180435977348 ) ) ;
#81354=EDGE_CURVE ( 'NONE', #32777, #104745, #117996, .T. ) ;
#81355=AXIS2_PLACEMENT_3D ( 'NONE', #7722, #95475, #125565 ) ;
#81356=DIRECTION ( 'NONE',  ( 0.000000000000000000, 1.000000000000000000, 0.000000000000000000 ) ) ;
#81357=EDGE_CURVE ( 'NONE', #37854, #53973, #22146, .T. ) ;
#81358=ORIENTED_EDGE ( 'NONE', *, *, #27989, .T. ) ;
#81359=ORIENTED_EDGE ( 'NONE', *, *, #41877, .F. ) ;
#81360=ORIENTED_EDGE ( 'NONE', *, *, #76862, .F. ) ;
#81361=EDGE_CURVE ( 'NONE', #77956, #128073, #65766, .T. ) ;
#81362=CARTESIAN_POINT ( 'NONE',  ( 8.749999999999953815, 12.50000000000000000, -2.165063509461101710 ) ) ;
#81363=ADVANCED_FACE ( 'NONE', ( #33252 ), #3091, .T. ) ;
#81364=AXIS2_PLACEMENT_3D ( 'NONE', #41192, #93492, #70623 ) ;
#81365=EDGE_CURVE ( 'NONE', #75566, #40560, #72525, .T. ) ;
#81366=DIRECTION ( 'NONE',  ( 0.000000000000000000, 0.000000000000000000, 1.000000000000000000 ) ) ;
#81367=SURFACE_STYLE_FILL_AREA ( #41449 ) ;
#81368=CARTESIAN_POINT ( 'NONE',  ( 14.59999999999989484, 12.50000000000000000, 0.6928203230275494784 ) ) ;
#81369=CARTESIAN_POINT ( 'NONE',  ( 4.799999999999937650, 12.50000000000000000, -3.918623584224389056 ) ) ;
#81370=CARTESIAN_POINT ( 'NONE',  ( -12.09999999999999609, 2.500000000000000000, -4.430127018922199511 ) ) ;
#81371=CARTESIAN_POINT ( 'NONE',  ( 10.59999999999990905, 12.50000000000000000, 4.048810130592458201 ) ) ;
#81372=EDGE_CURVE ( 'NONE', #59884, #88341, #5128, .T. ) ;
#81373=ORIENTED_EDGE ( 'NONE', *, *, #74741, .F. ) ;
#81374=ADVANCED_FACE ( 'NONE', ( #43081 ), #38612, .T. ) ;
#81375=AXIS2_PLACEMENT_3D ( 'NONE', #39575, #128597, #121319 ) ;
#81376=DIRECTION ( 'NONE',  ( -0.000000000000000000, 1.000000000000000000, -0.000000000000000000 ) ) ;
#81377=EDGE_LOOP ( 'NONE', ( #10493, #33825 ) ) ;
#81378=AXIS2_PLACEMENT_3D ( 'NONE', #40652, #28882, #68791 ) ;
#81379=EDGE_LOOP ( 'NONE', ( #58876, #125826, #89541, #26749 ) ) ;
#81380=EDGE_LOOP ( 'NONE', ( #102037, #77467 ) ) ;
#81381=DIRECTION ( 'NONE',  ( -0.000000000000000000, -1.000000000000000000, -0.000000000000000000 ) ) ;
#81382=VERTEX_POINT ( 'NONE', #23395 ) ;
#81383=ORIENTED_EDGE ( 'NONE', *, *, #9051, .F. ) ;
#81384=EDGE_LOOP ( 'NONE', ( #100941, #115251, #92259, #74825 ) ) ;
#81385=VECTOR ( 'NONE', #74857, 1000.000000000000000 ) ;
#81386=CARTESIAN_POINT ( 'NONE',  ( 3.949999999999939782, 12.50000000000000000, 2.511473670974873507 ) ) ;
#81387=CONICAL_SURFACE ( 'NONE', #10265, 0.1000000000000000472, 0.003490658503988666988 ) ;
#81388=DIRECTION ( 'NONE',  ( -0.000000000000000000, 1.000000000000000000, -0.000000000000000000 ) ) ;
#81389=CARTESIAN_POINT ( 'NONE',  ( 15.39999999999989200, 12.50000000000000000, 0.6928203230275494784 ) ) ;
#81390=DIRECTION ( 'NONE',  ( 0.000000000000000000, 0.000000000000000000, 1.000000000000000000 ) ) ;
#81391=DIRECTION ( 'NONE',  ( 0.000000000000000000, -0.9999939076577903929, 0.003490651415223739937 ) ) ;
#81392=FACE_OUTER_BOUND ( 'NONE', #13105, .T. ) ;
#81394=ORIENTED_EDGE ( 'NONE', *, *, #100088, .F. ) ;
#81395=DIRECTION ( 'NONE',  ( 0.000000000000000000, 1.000000000000000000, 0.000000000000000000 ) ) ;
#81396=ORIENTED_EDGE ( 'NONE', *, *, #37475, .T. ) ;
#81398=DIRECTION ( 'NONE',  ( 0.000000000000000000, -0.000000000000000000, 1.000000000000000000 ) ) ;
#81399=VECTOR ( 'NONE', #99280, 1000.000000000000000 ) ;
#81400=ORIENTED_EDGE ( 'NONE', *, *, #56602, .T. ) ;
#81401=CARTESIAN_POINT ( 'NONE',  ( 0.1999999999999567124, 2.500000000000000000, -4.083716857408426826 ) ) ;
#81402=VERTEX_POINT ( 'NONE', #13574 ) ;
#81404=EDGE_CURVE ( 'NONE', #59320, #45275, #121597, .T. ) ;
#81405=DIRECTION ( 'NONE',  ( 0.000000000000000000, 1.000000000000000000, 0.000000000000000000 ) ) ;
#81406=EDGE_CURVE ( 'NONE', #74953, #4337, #30201, .T. ) ;
#81407=ORIENTED_EDGE ( 'NONE', *, *, #97529, .F. ) ;
#81408=EDGE_LOOP ( 'NONE', ( #91537, #39454 ) ) ;
#81410=CARTESIAN_POINT ( 'NONE',  ( -2.900000000000029221, 2.500000000000000000, -2.276824562219559311E-15 ) ) ;
#81412=CARTESIAN_POINT ( 'NONE',  ( 1.849999999999950573, 2.500000000000000000, -1.818653347947326138 ) ) ;
#81413=CIRCLE ( 'NONE', #52466, 0.06509327318403745899 ) ;
#81414=ADVANCED_FACE ( 'NONE', ( #71881 ), #55322, .T. ) ;
#81415=CARTESIAN_POINT ( 'NONE',  ( 10.84999999999990905, 2.500000000000000000, 2.757883832488649656 ) ) ;
#81416=ORIENTED_EDGE ( 'NONE', *, *, #25456, .F. ) ;
#81417=CARTESIAN_POINT ( 'NONE',  ( 7.949999999999922018, 2.500000000000000000, 6.595190528383296780 ) ) ;
#81418=ORIENTED_EDGE ( 'NONE', *, *, #36717, .T. ) ;
#81419=DIRECTION ( 'NONE',  ( 0.000000000000000000, 0.000000000000000000, 1.000000000000000000 ) ) ;
#81420=DIRECTION ( 'NONE',  ( 0.000000000000000000, 1.000000000000000000, 0.000000000000000000 ) ) ;
#81421=AXIS2_PLACEMENT_3D ( 'NONE', #31196, #1066, #31824 ) ;
#81422=CONICAL_SURFACE ( 'NONE', #98126, 0.1000000000000002554, 0.003490658503988666988 ) ;
#81423=FACE_OUTER_BOUND ( 'NONE', #101083, .T. ) ;
#81424=DIRECTION ( 'NONE',  ( -0.000000000000000000, 1.000000000000000000, -0.000000000000000000 ) ) ;
#81425=FACE_OUTER_BOUND ( 'NONE', #52528, .T. ) ;
#81426=FACE_OUTER_BOUND ( 'NONE', #69604, .T. ) ;
#81427=CARTESIAN_POINT ( 'NONE',  ( 5.399999999999932854, 2.500000000000000000, 5.022947341949748790 ) ) ;
#81428=EDGE_LOOP ( 'NONE', ( #43882, #5392, #35911, #92186 ) ) ;
#81429=AXIS2_PLACEMENT_3D ( 'NONE', #62290, #1413, #78226 ) ;
#81430=DIRECTION ( 'NONE',  ( 0.000000000000000000, 0.000000000000000000, 1.000000000000000000 ) ) ;
#81432=CARTESIAN_POINT ( 'NONE',  ( 0.7999999999999548583, 12.50000000000000000, 4.330127018922196314 ) ) ;
#81433=ORIENTED_EDGE ( 'NONE', *, *, #99081, .F. ) ;
#81434=DIRECTION ( 'NONE',  ( 0.000000000000000000, 0.000000000000000000, 1.000000000000000000 ) ) ;
#81436=ORIENTED_EDGE ( 'NONE', *, *, #43879, .T. ) ;
#81437=EDGE_LOOP ( 'NONE', ( #44472, #91673 ) ) ;
#81438=LINE ( 'NONE', #40220, #109508 ) ;
#81439=AXIS2_PLACEMENT_3D ( 'NONE', #38178, #108194, #8061 ) ;
#81440=ORIENTED_EDGE ( 'NONE', *, *, #44636, .F. ) ;
#81441=EDGE_CURVE ( 'NONE', #99852, #13428, #122268, .T. ) ;
#81442=CARTESIAN_POINT ( 'NONE',  ( 21.23528140090950345, -2.699413673072311948, -2.293764360948883141 ) ) ;
#81443=DIRECTION ( 'NONE',  ( 0.000000000000000000, 0.000000000000000000, 1.000000000000000000 ) ) ;
#81444=ORIENTED_EDGE ( 'NONE', *, *, #110104, .T. ) ;
#81445=CIRCLE ( 'NONE', #12474, 0.1000000000000002554 ) ;
#81446=DIRECTION ( 'NONE',  ( 0.000000000000000000, 1.000000000000000000, 0.000000000000000000 ) ) ;
#81447=DIRECTION ( 'NONE',  ( 0.000000000000000000, 1.000000000000000000, 0.000000000000000000 ) ) ;
#81448=EDGE_CURVE ( 'NONE', #121848, #23090, #73788, .T. ) ;
#81449=VECTOR ( 'NONE', #12643, 1000.000000000000000 ) ;
#81450=VERTEX_POINT ( 'NONE', #44329 ) ;
#81451=CIRCLE ( 'NONE', #56394, 0.1000000000000002554 ) ;
#81452=VECTOR ( 'NONE', #98250, 1000.000000000000000 ) ;
#81453=AXIS2_PLACEMENT_3D ( 'NONE', #124983, #24848, #16292 ) ;
#81454=EDGE_LOOP ( 'NONE', ( #18735, #6896 ) ) ;
#81455=ORIENTED_EDGE ( 'NONE', *, *, #65421, .F. ) ;
#81456=LINE ( 'NONE', #62472, #4426 ) ;
#81457=CARTESIAN_POINT ( 'NONE',  ( 11.69999999999990870, 12.50000000000000000, -4.330127018922201643 ) ) ;
#81458=DIRECTION ( 'NONE',  ( -0.000000000000000000, 1.000000000000000000, -0.000000000000000000 ) ) ;
#81459=EDGE_CURVE ( 'NONE', #109667, #123049, #128496, .T. ) ;
#81460=FACE_BOUND ( 'NONE', #103103, .T. ) ;
#81461=ORIENTED_EDGE ( 'NONE', *, *, #90882, .F. ) ;
#81462=CONICAL_SURFACE ( 'NONE', #45965, 0.1000000000000002554, 0.003490658503988666988 ) ;
#81463=DIRECTION ( 'NONE',  ( 0.000000000000000000, -0.000000000000000000, 1.000000000000000000 ) ) ;
#81464=DIRECTION ( 'NONE',  ( 0.000000000000000000, 0.000000000000000000, 1.000000000000000000 ) ) ;
#81465=ORIENTED_EDGE ( 'NONE', *, *, #111683, .T. ) ;
#81466=CIRCLE ( 'NONE', #54271, 0.09999999999999982514 ) ;
#81467=DIRECTION ( 'NONE',  ( 0.000000000000000000, 0.000000000000000000, 1.000000000000000000 ) ) ;
#81468=DIRECTION ( 'NONE',  ( 0.000000000000000000, 1.000000000000000000, 0.000000000000000000 ) ) ;
#81469=FACE_OUTER_BOUND ( 'NONE', #91833, .T. ) ;
#81470=CARTESIAN_POINT ( 'NONE',  ( 10.44999999999991047, 2.500000000000000000, -6.595190528383302109 ) ) ;
#81471=DIRECTION ( 'NONE',  ( -0.000000000000000000, -1.000000000000000000, -0.000000000000000000 ) ) ;
#81472=DIRECTION ( 'NONE',  ( 0.000000000000000000, 0.000000000000000000, 1.000000000000000000 ) ) ;
#81473=DIRECTION ( 'NONE',  ( -0.000000000000000000, 1.000000000000000000, -0.000000000000000000 ) ) ;
#81474=VECTOR ( 'NONE', #113952, 1000.000000000000000 ) ;
#81475=ORIENTED_EDGE ( 'NONE', *, *, #47803, .T. ) ;
#81476=ORIENTED_EDGE ( 'NONE', *, *, #114608, .F. ) ;
#81477=EDGE_LOOP ( 'NONE', ( #115866, #52787 ) ) ;
#81478=ORIENTED_EDGE ( 'NONE', *, *, #37766, .T. ) ;
#81479=CARTESIAN_POINT ( 'NONE',  ( 11.44999999999991047, 12.50000000000000000, 6.148780366869520009 ) ) ;
#81480=CARTESIAN_POINT ( 'NONE',  ( -4.150000000000024336, 2.500000000000000000, 1.572243186433545548 ) ) ;
#81481=ORIENTED_EDGE ( 'NONE', *, *, #110057, .F. ) ;
#81482=FACE_BOUND ( 'NONE', #1451, .T. ) ;
#81483=DIRECTION ( 'NONE',  ( -0.000000000000000000, 1.000000000000000000, -0.000000000000000000 ) ) ;
#81484=CARTESIAN_POINT ( 'NONE',  ( 1.649999999999951505, 12.50000000000000000, 1.407149913249508000 ) ) ;
#81485=CARTESIAN_POINT ( 'NONE',  ( 2.899999999999943956, 2.500000000000000000, 4.230127018922196669 ) ) ;
#81486=EDGE_CURVE ( 'NONE', #85725, #120306, #57372, .T. ) ;
#81487=DIRECTION ( 'NONE',  ( -0.000000000000000000, 1.000000000000000000, -0.000000000000000000 ) ) ;
#81488=DIRECTION ( 'NONE',  ( 0.000000000000000000, 0.000000000000000000, 1.000000000000000000 ) ) ;
#81489=CARTESIAN_POINT ( 'NONE',  ( 15.59999999999988951, 2.500000000000000000, 0.4464101615137735513 ) ) ;
#81490=FACE_OUTER_BOUND ( 'NONE', #93744, .T. ) ;
#81491=DIRECTION ( 'NONE',  ( 0.000000000000000000, 1.000000000000000000, 0.000000000000000000 ) ) ;
#81492=ADVANCED_FACE ( 'NONE', ( #94084 ), #126421, .T. ) ;
#81493=CARTESIAN_POINT ( 'NONE',  ( -14.59999999999998366, 2.500000000000000000, 0.7928203230275517877 ) ) ;
#81494=EDGE_LOOP ( 'NONE', ( #111431, #97047 ) ) ;
#81495=ADVANCED_FACE ( 'NONE', ( #21477 ), #57470, .T. ) ;
#81496=ORIENTED_EDGE ( 'NONE', *, *, #62858, .F. ) ;
#81497=ORIENTED_EDGE ( 'NONE', *, *, #119637, .T. ) ;
#81498=ORIENTED_EDGE ( 'NONE', *, *, #83299, .F. ) ;
#81499=VERTEX_POINT ( 'NONE', #112448 ) ;
#81500=EDGE_LOOP ( 'NONE', ( #36530, #17481 ) ) ;
#81501=EDGE_CURVE ( 'NONE', #72150, #33066, #9441, .T. ) ;
#81503=ADVANCED_FACE ( 'NONE', ( #96633 ), #1023, .T. ) ;
#81504=CIRCLE ( 'NONE', #27120, 0.06509327318403745899 ) ;
#81505=ADVANCED_FACE ( 'NONE', ( #46261 ), #47011, .T. ) ;
#81506=EDGE_LOOP ( 'NONE', ( #80024, #74484 ) ) ;
#81507=VECTOR ( 'NONE', #43597, 1000.000000000000000 ) ;
#81508=CARTESIAN_POINT ( 'NONE',  ( -1.450000000000035039, 12.50000000000000000, -6.841600689897077814 ) ) ;
#81509=AXIS2_PLACEMENT_3D ( 'NONE', #58604, #49437, #68402 ) ;
#81510=ADVANCED_FACE ( 'NONE', ( #6958 ), #95119, .T. ) ;
#81511=CARTESIAN_POINT ( 'NONE',  ( 4.149999999999939959, 2.500000000000000000, 2.757883832488649656 ) ) ;
#81513=CARTESIAN_POINT ( 'NONE',  ( 14.34999999999989306, 2.500000000000000000, -2.511473670974877948 ) ) ;
#81514=ORIENTED_EDGE ( 'NONE', *, *, #60211, .F. ) ;
#81515=CARTESIAN_POINT ( 'NONE',  ( -4.600000000000025402, 2.500000000000000000, 4.330127018922196314 ) ) ;
#81516=ADVANCED_FACE ( 'NONE', ( #14844 ), #126511, .T. ) ;
#81517=AXIS2_PLACEMENT_3D ( 'NONE', #74805, #12641, #12006 ) ;
#81518=EDGE_LOOP ( 'NONE', ( #112568, #6634, #127377, #102837 ) ) ;
#81519=ORIENTED_EDGE ( 'NONE', *, *, #63017, .F. ) ;
#81520=FACE_OUTER_BOUND ( 'NONE', #119325, .T. ) ;
#81521=DIRECTION ( 'NONE',  ( 0.000000000000000000, 1.000000000000000000, 0.000000000000000000 ) ) ;
#81522=CARTESIAN_POINT ( 'NONE',  ( 11.69999999999990870, 12.50000000000000000, 4.330127018922196314 ) ) ;
#81523=VERTEX_POINT ( 'NONE', #95375 ) ;
#81524=EDGE_LOOP ( 'NONE', ( #45731, #31404, #113136, #903 ) ) ;
#81525=LINE ( 'NONE', #110335, #61068 ) ;
#81526=CARTESIAN_POINT ( 'NONE',  ( 9.349999999999919709, 12.50000000000000000, -6.841600689897078702 ) ) ;
#81527=DIRECTION ( 'NONE',  ( 0.000000000000000000, 1.000000000000000000, 0.000000000000000000 ) ) ;
#81528=CARTESIAN_POINT ( 'NONE',  ( 14.99999999999989164, 2.500000000000000000, 0.6928203230275494784 ) ) ;
#81529=ORIENTED_EDGE ( 'NONE', *, *, #12933, .T. ) ;
#81530=DIRECTION ( 'NONE',  ( 0.000000000000000000, 0.000000000000000000, 1.000000000000000000 ) ) ;
#81531=VERTEX_POINT ( 'NONE', #96016 ) ;
#81532=DIRECTION ( 'NONE',  ( 0.000000000000000000, 0.000000000000000000, 1.000000000000000000 ) ) ;
#81533=AXIS2_PLACEMENT_3D ( 'NONE', #12443, #52381, #694 ) ;
#81534=AXIS2_PLACEMENT_3D ( 'NONE', #54585, #36272, #128534 ) ;
#81535=ORIENTED_EDGE ( 'NONE', *, *, #48756, .F. ) ;
#81536=DIRECTION ( 'NONE',  ( 0.000000000000000000, 0.000000000000000000, -1.000000000000000000 ) ) ;
#81537=DIRECTION ( 'NONE',  ( 0.000000000000000000, 0.000000000000000000, -1.000000000000000000 ) ) ;
#81538=CARTESIAN_POINT ( 'NONE',  ( 9.349999999999919709, 12.50000000000000000, -6.148780366869526226 ) ) ;
#81539=CARTESIAN_POINT ( 'NONE',  ( 13.94999999999989271, 2.500000000000000000, -1.818653347947326138 ) ) ;
#81540=LINE ( 'NONE', #80257, #93970 ) ;
#81541=ORIENTED_EDGE ( 'NONE', *, *, #115309, .F. ) ;
#81542=VECTOR ( 'NONE', #81734, 1000.000000000000000 ) ;
#81543=CARTESIAN_POINT ( 'NONE',  ( -11.64999999999999680, 12.50000000000000000, 5.867463478539781896 ) ) ;
#81544=ADVANCED_FACE ( 'NONE', ( #125470 ), #13532, .T. ) ;
#81545=DIRECTION ( 'NONE',  ( -0.000000000000000000, 1.000000000000000000, -0.000000000000000000 ) ) ;
#81546=ORIENTED_EDGE ( 'NONE', *, *, #19214, .F. ) ;
#81547=VERTEX_POINT ( 'NONE', #54787 ) ;
#81548=ORIENTED_EDGE ( 'NONE', *, *, #111782, .T. ) ;
#81549=CARTESIAN_POINT ( 'NONE',  ( 11.24999999999990585, 2.500000000000000000, 2.857883832488649301 ) ) ;
#81550=CARTESIAN_POINT ( 'NONE',  ( -7.499999999999980460, 2.500000000000000000, -4.430127018922202176 ) ) ;
#81552=AXIS2_PLACEMENT_3D ( 'NONE', #46511, #36721, #59436 ) ;
#81553=CARTESIAN_POINT ( 'NONE',  ( 4.349999999999941025, 2.500000000000000000, -1.818653347947326138 ) ) ;
#81554=DIRECTION ( 'NONE',  ( 0.000000000000000000, 0.000000000000000000, 1.000000000000000000 ) ) ;
#81555=EDGE_CURVE ( 'NONE', #8118, #54678, #5215, .T. ) ;
#81556=VECTOR ( 'NONE', #61785, 1000.000000000000000 ) ;
#81558=CARTESIAN_POINT ( 'NONE',  ( -10.60000000000000142, 2.500000000000000000, 4.676537180435972552 ) ) ;
#81559=CARTESIAN_POINT ( 'NONE',  ( -4.150000000000024336, 2.500000000000000000, -2.065063509461102065 ) ) ;
#81561=VERTEX_POINT ( 'NONE', #45641 ) ;
#81562=CIRCLE ( 'NONE', #20927, 0.1000000000000000472 ) ;
#81563=DIRECTION ( 'NONE',  ( 0.000000000000000000, 0.000000000000000000, -1.000000000000000000 ) ) ;
#81564=DIRECTION ( 'NONE',  ( 0.000000000000000000, 1.000000000000000000, 0.000000000000000000 ) ) ;
#81565=DIRECTION ( 'NONE',  ( 0.000000000000000000, -0.9999939076577903929, 0.003490651415223739937 ) ) ;
#81566=CARTESIAN_POINT ( 'NONE',  ( -0.4000000000000392131, 2.500000000000000000, -4.330127018922201643 ) ) ;
#81567=ORIENTED_EDGE ( 'NONE', *, *, #72956, .T. ) ;
#81568=DIRECTION ( 'NONE',  ( -0.000000000000000000, 1.000000000000000000, -0.000000000000000000 ) ) ;
#81569=DIRECTION ( 'NONE',  ( 0.000000000000000000, 0.000000000000000000, 1.000000000000000000 ) ) ;
#81570=DIRECTION ( 'NONE',  ( -4.274815082592931898E-19, -0.9999939076577903929, -0.003490651415223739937 ) ) ;
#81571=ORIENTED_EDGE ( 'NONE', *, *, #76130, .T. ) ;
#81572=VERTEX_POINT ( 'NONE', #76384 ) ;
#81573=DIRECTION ( 'NONE',  ( -4.274815082592931898E-19, -0.9999939076577903929, -0.003490651415223739937 ) ) ;
#81574=ADVANCED_FACE ( 'NONE', ( #107107 ), #85547, .T. ) ;
#81575=VERTEX_POINT ( 'NONE', #86166 ) ;
#81576=ORIENTED_EDGE ( 'NONE', *, *, #56947, .F. ) ;
#81577=DIRECTION ( 'NONE',  ( 0.000000000000000000, 0.000000000000000000, -1.000000000000000000 ) ) ;
#81578=CIRCLE ( 'NONE', #58608, 0.1000000000000000472 ) ;
#81579=CARTESIAN_POINT ( 'NONE',  ( 20.37025966759639672, 0.6621301594404709334, -4.188616773932404946 ) ) ;
#81580=LINE ( 'NONE', #51496, #10781 ) ;
#81581=DIRECTION ( 'NONE',  ( 0.000000000000000000, 0.000000000000000000, 1.000000000000000000 ) ) ;
#81582=ADVANCED_FACE ( 'NONE', ( #67163 ), #36475, .T. ) ;
#81583=EDGE_LOOP ( 'NONE', ( #22117, #24900, #39462 ) ) ;
#81584=AXIS2_PLACEMENT_3D ( 'NONE', #21867, #1554, #110857 ) ;
#81586=DIRECTION ( 'NONE',  ( -0.000000000000000000, -1.000000000000000000, -0.000000000000000000 ) ) ;
#81587=EDGE_LOOP ( 'NONE', ( #88294, #119625 ) ) ;
#81588=ADVANCED_FACE ( 'NONE', ( #75719 ), #44947, .T. ) ;
#81589=CARTESIAN_POINT ( 'NONE',  ( -13.54999999999998828, 2.500000000000000000, -2.611473670974875372 ) ) ;
#81591=ADVANCED_FACE ( 'NONE', ( #65246 ), #3184, .T. ) ;
#81592=ORIENTED_EDGE ( 'NONE', *, *, #63017, .T. ) ;
#81593=ORIENTED_EDGE ( 'NONE', *, *, #58306, .F. ) ;
#81595=ORIENTED_EDGE ( 'NONE', *, *, #10675, .T. ) ;
#81597=CARTESIAN_POINT ( 'NONE',  ( -6.250000000000019540, 2.500000000000000000, -2.957883832488653830 ) ) ;
#81598=DIRECTION ( 'NONE',  ( -0.000000000000000000, -1.000000000000000000, -0.000000000000000000 ) ) ;
#81599=DIRECTION ( 'NONE',  ( 0.000000000000000000, 0.000000000000000000, -1.000000000000000000 ) ) ;
#81600=ADVANCED_FACE ( 'NONE', ( #84903 ), #106479, .T. ) ;
#81601=FACE_BOUND ( 'NONE', #115061, .T. ) ;
#81602=ORIENTED_EDGE ( 'NONE', *, *, #56234, .T. ) ;
#81603=CARTESIAN_POINT ( 'NONE',  ( 11.64999999999990798, 2.500000000000000000, 7.088010851410848190 ) ) ;
#81605=LINE ( 'NONE', #31871, #67806 ) ;
#81606=CARTESIAN_POINT ( 'NONE',  ( 3.549999999999941203, 12.50000000000000000, 6.148780366869520897 ) ) ;
#81607=CARTESIAN_POINT ( 'NONE',  ( -4.350000000000023626, 12.50000000000000000, 1.818653347947321475 ) ) ;
#81608=FACE_OUTER_BOUND ( 'NONE', #70507, .T. ) ;
#81610=AXIS2_PLACEMENT_3D ( 'NONE', #124351, #115133, #102757 ) ;
#81611=CIRCLE ( 'NONE', #48175, 0.1000000000000002554 ) ;
#81612=DIRECTION ( 'NONE',  ( -0.000000000000000000, 1.000000000000000000, -0.000000000000000000 ) ) ;
#81613=ORIENTED_EDGE ( 'NONE', *, *, #88684, .T. ) ;
#81614=VERTEX_POINT ( 'NONE', #27264 ) ;
#81615=ORIENTED_EDGE ( 'NONE', *, *, #94855, .T. ) ;
#81616=ORIENTED_EDGE ( 'NONE', *, *, #18127, .T. ) ;
#81617=ORIENTED_EDGE ( 'NONE', *, *, #61057, .T. ) ;
#81618=DIRECTION ( 'NONE',  ( 0.000000000000000000, 1.000000000000000000, 0.000000000000000000 ) ) ;
#81619=CARTESIAN_POINT ( 'NONE',  ( -12.69999999999999041, 2.500000000000000000, 3.983716857408420964 ) ) ;
#81620=ORIENTED_EDGE ( 'NONE', *, *, #125952, .T. ) ;
#81621=FACE_BOUND ( 'NONE', #119952, .T. ) ;
#81622=CARTESIAN_POINT ( 'NONE',  ( 5.649999999999934630, 2.500000000000000000, -1.918653347947325782 ) ) ;
#81623=ADVANCED_FACE ( 'NONE', ( #35181 ), #86706, .T. ) ;
#81624=ORIENTED_EDGE ( 'NONE', *, *, #75287, .T. ) ;
#81625=CARTESIAN_POINT ( 'NONE',  ( -9.800000000000006040, 2.500000000000000000, -4.676537180435974328 ) ) ;
#81626=DIRECTION ( 'NONE',  ( -0.000000000000000000, 1.000000000000000000, -0.000000000000000000 ) ) ;
#81627=DIRECTION ( 'NONE',  ( 0.000000000000000000, 1.000000000000000000, 0.000000000000000000 ) ) ;
#81629=ORIENTED_EDGE ( 'NONE', *, *, #92381, .F. ) ;
#81630=FACE_OUTER_BOUND ( 'NONE', #99459, .T. ) ;
#81631=EDGE_CURVE ( 'NONE', #50586, #10571, #105833, .T. ) ;
#81632=VECTOR ( 'NONE', #22986, 1000.000000000000000 ) ;
#81633=ORIENTED_EDGE ( 'NONE', *, *, #87845, .F. ) ;
#81634=B_SPLINE_SURFACE_WITH_KNOTS ( 'NONE', 3, 1, ( 
 ( #100517, #10830 ),
 ( #90709, #1037 ),
 ( #23912, #103755 ),
 ( #64459, #82179 ),
 ( #114218, #121444 ),
 ( #33100, #33717 ),
 ( #122111, #24543 ),
 ( #54011, #72372 ),
 ( #93286, #104394 ),
 ( #103102, #42261 ),
 ( #112924, #63833 ),
 ( #74298, #62550 ),
 ( #31795, #73630 ),
 ( #42927, #12132 ),
 ( #14698, #124028 ),
 ( #111644, #52081 ),
 ( #14055, #84095 ),
 ( #102464, #54632 ) ),
 .UNSPECIFIED., .F., .F., .F.,
 ( 4, 2, 2, 2, 2, 2, 2, 2, 4 ),
 ( 2, 2 ),
 ( 0.000000000000000000, 0.1249999999999999445, 0.2499999999999998890, 0.3749999999999999445, 0.5000000000000000000, 0.6250000000000000000, 0.7500000000000001110, 0.8750000000000000000, 1.000000000000000000 ),
 ( 0.000000000000000000, 1.000000000000000000 ),
 .UNSPECIFIED. ) ;
#81635=VERTEX_POINT ( 'NONE', #71545 ) ;
#81636=ORIENTED_EDGE ( 'NONE', *, *, #39741, .F. ) ;
#81637=ADVANCED_FACE ( 'NONE', ( #101667 ), #92476, .T. ) ;
#81639=DIRECTION ( 'NONE',  ( 0.000000000000000000, -0.000000000000000000, 1.000000000000000000 ) ) ;
#81640=EDGE_CURVE ( 'NONE', #31627, #181, #11490, .T. ) ;
#81641=ORIENTED_EDGE ( 'NONE', *, *, #21665, .F. ) ;
#81642=CARTESIAN_POINT ( 'NONE',  ( -7.499999999999976907, 12.50000000000000000, 4.395220292106234439 ) ) ;
#81643=CIRCLE ( 'NONE', #77441, 0.09999999999999982514 ) ;
#81644=EDGE_CURVE ( 'NONE', #111547, #102327, #2810, .T. ) ;
#81645=LINE ( 'NONE', #12883, #28126 ) ;
#81646=CARTESIAN_POINT ( 'NONE',  ( 10.19999999999991580, 2.500000000000000000, -0.3464101615137783474 ) ) ;
#81647=DIRECTION ( 'NONE',  ( -0.000000000000000000, 1.000000000000000000, -0.000000000000000000 ) ) ;
#81648=EDGE_CURVE ( 'NONE', #16181, #118050, #70076, .T. ) ;
#81649=DIRECTION ( 'NONE',  ( 0.000000000000000000, 1.000000000000000000, 0.000000000000000000 ) ) ;
#81650=ORIENTED_EDGE ( 'NONE', *, *, #101590, .T. ) ;
#81651=DIRECTION ( 'NONE',  ( 0.000000000000000000, 0.000000000000000000, 1.000000000000000000 ) ) ;
#81652=EDGE_LOOP ( 'NONE', ( #124645, #54487 ) ) ;
#81653=DIRECTION ( 'NONE',  ( -0.000000000000000000, -1.000000000000000000, -0.000000000000000000 ) ) ;
#81654=EDGE_CURVE ( 'NONE', #40083, #126577, #30293, .T. ) ;
#81655=EDGE_CURVE ( 'NONE', #6702, #52447, #15672, .T. ) ;
#81656=ORIENTED_EDGE ( 'NONE', *, *, #85308, .T. ) ;
#81657=DIRECTION ( 'NONE',  ( 0.000000000000000000, -0.9999939076577903929, 0.003490651415223739937 ) ) ;
#81658=ORIENTED_EDGE ( 'NONE', *, *, #77370, .T. ) ;
#81659=DIRECTION ( 'NONE',  ( -0.000000000000000000, 1.000000000000000000, -0.000000000000000000 ) ) ;
#81660=DIRECTION ( 'NONE',  ( 0.000000000000000000, 0.000000000000000000, -1.000000000000000000 ) ) ;
#81661=DIRECTION ( 'NONE',  ( 0.000000000000000000, -0.9999939076577903929, 0.003490651415223739937 ) ) ;
#81662=DIRECTION ( 'NONE',  ( 0.000000000000000000, 0.000000000000000000, 1.000000000000000000 ) ) ;
#81664=VERTEX_POINT ( 'NONE', #21155 ) ;
#81665=ORIENTED_EDGE ( 'NONE', *, *, #104429, .F. ) ;
#81666=EDGE_LOOP ( 'NONE', ( #72526, #127490 ) ) ;
#81667=CARTESIAN_POINT ( 'NONE',  ( -5.200000000000020606, 2.500000000000000000, 3.983716857408420964 ) ) ;
#81669=VECTOR ( 'NONE', #119204, 1000.000000000000000 ) ;
#81671=EDGE_LOOP ( 'NONE', ( #111790, #129523, #129042, #41794 ) ) ;
#81672=ORIENTED_EDGE ( 'NONE', *, *, #22407, .T. ) ;
#81673=ORIENTED_EDGE ( 'NONE', *, *, #127487, .T. ) ;
#81674=CIRCLE ( 'NONE', #35708, 0.09999999999999982514 ) ;
#81675=CONICAL_SURFACE ( 'NONE', #25221, 0.1000000000000000056, 0.003490658503988666988 ) ;
#81676=DIRECTION ( 'NONE',  ( 0.000000000000000000, 0.000000000000000000, 1.000000000000000000 ) ) ;
#81677=EDGE_LOOP ( 'NONE', ( #43846, #108823 ) ) ;
#81678=DIRECTION ( 'NONE',  ( 0.000000000000000000, 0.000000000000000000, 1.000000000000000000 ) ) ;
#81679=DIRECTION ( 'NONE',  ( 0.000000000000000000, 0.000000000000000000, -1.000000000000000000 ) ) ;
#81680=AXIS2_PLACEMENT_3D ( 'NONE', #119897, #71418, #69492 ) ;
#81681=DIRECTION ( 'NONE',  ( -0.000000000000000000, -1.000000000000000000, -0.000000000000000000 ) ) ;
#81682=FACE_OUTER_BOUND ( 'NONE', #59847, .T. ) ;
#81683=DIRECTION ( 'NONE',  ( 0.000000000000000000, 0.000000000000000000, 1.000000000000000000 ) ) ;
#81684=CARTESIAN_POINT ( 'NONE',  ( 8.149999999999923972, 2.500000000000000000, 2.511473670974873507 ) ) ;
#81685=LINE ( 'NONE', #112453, #92785 ) ;
#81686=CIRCLE ( 'NONE', #50383, 0.09999999999999982514 ) ;
#81687=DIRECTION ( 'NONE',  ( 0.000000000000000000, 0.000000000000000000, 1.000000000000000000 ) ) ;
#81688=EDGE_LOOP ( 'NONE', ( #62627, #60919, #115952, #13963 ) ) ;
#81689=FACE_OUTER_BOUND ( 'NONE', #4276, .T. ) ;
#81690=CARTESIAN_POINT ( 'NONE',  ( 26.75237029038351366, -2.962322469583595907, 2.722363819585612355 ) ) ;
#81691=ORIENTED_EDGE ( 'NONE', *, *, #60800, .F. ) ;
#81692=VERTEX_POINT ( 'NONE', #42100 ) ;
#81694=LINE ( 'NONE', #41157, #53192 ) ;
#81695=CARTESIAN_POINT ( 'NONE',  ( 9.799999999999913669, 2.500000000000000000, 4.676537180435972552 ) ) ;
#81696=CARTESIAN_POINT ( 'NONE',  ( -1.050000000000037792, 2.500000000000000000, 1.918653347947321564 ) ) ;
#81697=DIRECTION ( 'NONE',  ( 0.000000000000000000, 0.000000000000000000, 1.000000000000000000 ) ) ;
#81698=ADVANCED_FACE ( 'NONE', ( #67839 ), #69990, .T. ) ;
#81699=CARTESIAN_POINT ( 'NONE',  ( -1.250000000000037526, 2.500000000000000000, -1.472243186433550122 ) ) ;
#81700=DIRECTION ( 'NONE',  ( 0.000000000000000000, 0.000000000000000000, 1.000000000000000000 ) ) ;
#81701=DIRECTION ( 'NONE',  ( 0.000000000000000000, 0.000000000000000000, 1.000000000000000000 ) ) ;
#81702=DIRECTION ( 'NONE',  ( 0.000000000000000000, -0.9999939076577903929, 0.003490651415223739937 ) ) ;
#81703=AXIS2_PLACEMENT_3D ( 'NONE', #88457, #89117, #107470 ) ;
#81704=ORIENTED_EDGE ( 'NONE', *, *, #66899, .F. ) ;
#81705=VECTOR ( 'NONE', #12770, 1000.000000000000000 ) ;
#81706=ORIENTED_EDGE ( 'NONE', *, *, #11738, .F. ) ;
#81707=ORIENTED_EDGE ( 'NONE', *, *, #73771, .T. ) ;
#81708=ORIENTED_EDGE ( 'NONE', *, *, #85591, .F. ) ;
#81710=FACE_OUTER_BOUND ( 'NONE', #121000, .T. ) ;
#81711=VECTOR ( 'NONE', #14122, 1000.000000000000000 ) ;
#81712=AXIS2_PLACEMENT_3D ( 'NONE', #11172, #18427, #51128 ) ;
#81713=EDGE_LOOP ( 'NONE', ( #50961, #82193, #49547, #28485 ) ) ;
#81714=FACE_OUTER_BOUND ( 'NONE', #122783, .T. ) ;
#81715=DIRECTION ( 'NONE',  ( -0.000000000000000000, 1.000000000000000000, -0.000000000000000000 ) ) ;
#81716=FACE_OUTER_BOUND ( 'NONE', #5230, .T. ) ;
#81717=CARTESIAN_POINT ( 'NONE',  ( -0.8500000000000390576, 2.500000000000000000, -2.165063509461101710 ) ) ;
#81718=ORIENTED_EDGE ( 'NONE', *, *, #101180, .T. ) ;
#81719=DIRECTION ( 'NONE',  ( 0.000000000000000000, -0.000000000000000000, 1.000000000000000000 ) ) ;
#81720=DIRECTION ( 'NONE',  ( -4.274815082592931898E-19, -0.9999939076577903929, -0.003490651415223739937 ) ) ;
#81721=AXIS2_PLACEMENT_3D ( 'NONE', #2512, #60820, #42479 ) ;
#81723=AXIS2_PLACEMENT_3D ( 'NONE', #32528, #82902, #70491 ) ;
#81724=ORIENTED_EDGE ( 'NONE', *, *, #75338, .T. ) ;
#81725=ORIENTED_EDGE ( 'NONE', *, *, #120745, .F. ) ;
#81726=ORIENTED_EDGE ( 'NONE', *, *, #84843, .T. ) ;
#81727=FACE_OUTER_BOUND ( 'NONE', #58037, .T. ) ;
#81728=CONICAL_SURFACE ( 'NONE', #106771, 0.1000000000000002554, 0.003490658503988666988 ) ;
#81729=DIRECTION ( 'NONE',  ( -0.000000000000000000, 1.000000000000000000, -0.000000000000000000 ) ) ;
#81731=ADVANCED_FACE ( 'NONE', ( #107767 ), #70915, .T. ) ;
#81732=VERTEX_POINT ( 'NONE', #82012 ) ;
#81733=AXIS2_PLACEMENT_3D ( 'NONE', #73559, #4171, #42862 ) ;
#81734=DIRECTION ( 'NONE',  ( 0.000000000000000000, -0.9999939076577903929, 0.003490651415223739937 ) ) ;
#81735=ORIENTED_EDGE ( 'NONE', *, *, #30790, .F. ) ;
#81736=DIRECTION ( 'NONE',  ( 0.000000000000000000, -0.000000000000000000, 1.000000000000000000 ) ) ;
#81737=DIRECTION ( 'NONE',  ( 0.000000000000000000, 0.000000000000000000, 1.000000000000000000 ) ) ;
#81738=EDGE_CURVE ( 'NONE', #76276, #29239, #2158, .T. ) ;
#81739=DIRECTION ( 'NONE',  ( 0.000000000000000000, -0.000000000000000000, 1.000000000000000000 ) ) ;
#81740=FACE_OUTER_BOUND ( 'NONE', #70342, .T. ) ;
#81741=EDGE_CURVE ( 'NONE', #37231, #70629, #112132, .T. ) ;
#81742=VERTEX_POINT ( 'NONE', #22478 ) ;
#81743=VERTEX_POINT ( 'NONE', #51294 ) ;
#81744=ADVANCED_FACE ( 'NONE', ( #28568 ), #12617, .T. ) ;
#81745=EDGE_CURVE ( 'NONE', #127958, #80681, #20529, .T. ) ;
#81746=ORIENTED_EDGE ( 'NONE', *, *, #49869, .F. ) ;
#81747=DIRECTION ( 'NONE',  ( 0.000000000000000000, 1.000000000000000000, 0.000000000000000000 ) ) ;
#81748=DIRECTION ( 'NONE',  ( 0.000000000000000000, 1.000000000000000000, 0.000000000000000000 ) ) ;
#81750=FACE_BOUND ( 'NONE', #97876, .T. ) ;
#81751=DIRECTION ( 'NONE',  ( 0.000000000000000000, -0.000000000000000000, 1.000000000000000000 ) ) ;
#81752=DIRECTION ( 'NONE',  ( 0.000000000000000000, 0.000000000000000000, 1.000000000000000000 ) ) ;
#81753=DIRECTION ( 'NONE',  ( 0.000000000000000000, -0.000000000000000000, 1.000000000000000000 ) ) ;
#81754=AXIS2_PLACEMENT_3D ( 'NONE', #45805, #5211, #87002 ) ;
#81755=CIRCLE ( 'NONE', #83906, 0.06509327318403745899 ) ;
#81756=DIRECTION ( 'NONE',  ( 0.000000000000000000, -0.000000000000000000, 1.000000000000000000 ) ) ;
#81757=AXIS2_PLACEMENT_3D ( 'NONE', #101666, #59833, #81390 ) ;
#81758=CARTESIAN_POINT ( 'NONE',  ( -11.44999999999999751, 2.500000000000000000, 6.148780366869520897 ) ) ;
#81759=DIRECTION ( 'NONE',  ( 0.000000000000000000, 1.000000000000000000, 0.000000000000000000 ) ) ;
#81760=ORIENTED_EDGE ( 'NONE', *, *, #16789, .T. ) ;
#81761=CARTESIAN_POINT ( 'NONE',  ( 10.64999999999991331, 2.500000000000000000, -1.818653347947325916 ) ) ;
#81762=AXIS2_PLACEMENT_3D ( 'NONE', #23624, #52437, #2042 ) ;
#81763=DIRECTION ( 'NONE',  ( 0.000000000000000000, -0.9999939076577903929, 0.003490651415223739937 ) ) ;
#81764=VERTEX_POINT ( 'NONE', #18091 ) ;
#81765=VERTEX_POINT ( 'NONE', #97943 ) ;
#81766=CONICAL_SURFACE ( 'NONE', #90161, 0.1000000000000002554, 0.003490658503988666988 ) ;
#81767=CARTESIAN_POINT ( 'NONE',  ( -5.400000000000019895, 2.500000000000000000, 3.737306695894644371 ) ) ;
#81768=DIRECTION ( 'NONE',  ( 0.000000000000000000, 0.000000000000000000, 1.000000000000000000 ) ) ;
#81769=FACE_BOUND ( 'NONE', #75710, .T. ) ;
#81770=CARTESIAN_POINT ( 'NONE',  ( 7.899999999999923084, 2.500000000000000000, 0.5928203230275495006 ) ) ;
#81772=DIRECTION ( 'NONE',  ( 0.000000000000000000, 0.000000000000000000, 1.000000000000000000 ) ) ;
#81773=EDGE_CURVE ( 'NONE', #103770, #11509, #36646, .T. ) ;
#81775=ORIENTED_EDGE ( 'NONE', *, *, #64490, .F. ) ;
#81776=CARTESIAN_POINT ( 'NONE',  ( 11.44999999999991047, 2.500000000000000000, -2.611473670974877592 ) ) ;
#81777=CARTESIAN_POINT ( 'NONE',  ( -4.200000000000029488, 12.50000000000000000, -4.330127018922201643 ) ) ;
#81778=EDGE_CURVE ( 'NONE', #47295, #113860, #63727, .T. ) ;
#81779=ORIENTED_EDGE ( 'NONE', *, *, #79092, .F. ) ;
#81780=EDGE_CURVE ( 'NONE', #39986, #41483, #7268, .T. ) ;
#81781=CARTESIAN_POINT ( 'NONE',  ( -0.4500000000000397571, 2.500000000000000000, -6.595190528383302109 ) ) ;
#81782=DIRECTION ( 'NONE',  ( -0.000000000000000000, 1.000000000000000000, -0.000000000000000000 ) ) ;
#81783=EDGE_CURVE ( 'NONE', #106452, #39808, #105676, .T. ) ;
#81784=CIRCLE ( 'NONE', #90098, 0.06509327318403745899 ) ;
#81785=AXIS2_PLACEMENT_3D ( 'NONE', #61096, #89904, #69621 ) ;
#81786=EDGE_LOOP ( 'NONE', ( #64558, #91558, #124934, #22656 ) ) ;
#81787=DIRECTION ( 'NONE',  ( -0.000000000000000000, 1.000000000000000000, -0.000000000000000000 ) ) ;
#81788=LINE ( 'NONE', #71997, #53912 ) ;
#81789=CARTESIAN_POINT ( 'NONE',  ( -7.500000000000001776, 2.500000000000000000, 1.734723475976807094E-15 ) ) ;
#81790=EDGE_CURVE ( 'NONE', #124254, #43141, #105528, .T. ) ;
#81791=EDGE_LOOP ( 'NONE', ( #62753, #60442, #20174, #46966 ) ) ;
#81792=ORIENTED_EDGE ( 'NONE', *, *, #27956, .F. ) ;
#81793=ADVANCED_FACE ( 'NONE', ( #35507 ), #109883, .T. ) ;
#81794=DIRECTION ( 'NONE',  ( 0.000000000000000000, 1.000000000000000000, 0.000000000000000000 ) ) ;
#81795=VECTOR ( 'NONE', #9142, 1000.000000000000000 ) ;
#81796=ADVANCED_FACE ( 'NONE', ( #53849 ), #47104, .T. ) ;
#81797=ORIENTED_EDGE ( 'NONE', *, *, #110352, .T. ) ;
#81798=CARTESIAN_POINT ( 'NONE',  ( -13.34999999999999076, 12.50000000000000000, 1.407149913249511997 ) ) ;
#81799=CONICAL_SURFACE ( 'NONE', #92264, 0.1000000000000002554, 0.003490658503988666988 ) ;
#81800=CARTESIAN_POINT ( 'NONE',  ( 1.899999999999951283, 12.50000000000000000, -4.676537180435977881 ) ) ;
#81801=ADVANCED_FACE ( 'NONE', ( #115305 ), #57562, .T. ) ;
#81802=EDGE_CURVE ( 'NONE', #62761, #93687, #107725, .T. ) ;
#81803=LINE ( 'NONE', #35782, #92751 ) ;
#81804=EDGE_LOOP ( 'NONE', ( #5431, #15325 ) ) ;
#81805=CARTESIAN_POINT ( 'NONE',  ( 11.24999999999990941, 2.500000000000000000, -1.572243186433550211 ) ) ;
#81806=DIRECTION ( 'NONE',  ( 0.000000000000000000, 0.000000000000000000, 1.000000000000000000 ) ) ;
#81807=DIRECTION ( 'NONE',  ( -0.000000000000000000, -1.000000000000000000, -0.000000000000000000 ) ) ;
#81808=FACE_OUTER_BOUND ( 'NONE', #24656, .T. ) ;
#81809=FACE_OUTER_BOUND ( 'NONE', #101515, .T. ) ;
#81810=DIRECTION ( 'NONE',  ( 0.000000000000000000, 0.000000000000000000, 1.000000000000000000 ) ) ;
#81811=ADVANCED_FACE ( 'NONE', ( #122591 ), #72241, .T. ) ;
#81812=AXIS2_PLACEMENT_3D ( 'NONE', #39755, #107822, #79647 ) ;
#81813=EDGE_LOOP ( 'NONE', ( #115777, #506, #1137, #65283 ) ) ;
#81814=AXIS2_PLACEMENT_3D ( 'NONE', #8821, #108323, #107020 ) ;
#81815=ORIENTED_EDGE ( 'NONE', *, *, #25019, .F. ) ;
#81816=DIRECTION ( 'NONE',  ( 0.000000000000000000, 1.000000000000000000, 0.000000000000000000 ) ) ;
#81817=ORIENTED_EDGE ( 'NONE', *, *, #105742, .F. ) ;
#81819=CONICAL_SURFACE ( 'NONE', #37914, 0.1000000000000002554, 0.003490658503988666988 ) ;
#81820=EDGE_LOOP ( 'NONE', ( #86532, #128397 ) ) ;
#81821=VERTEX_POINT ( 'NONE', #45328 ) ;
#81822=ORIENTED_EDGE ( 'NONE', *, *, #102143, .F. ) ;
#81823=DIRECTION ( 'NONE',  ( 0.000000000000000000, -0.000000000000000000, 1.000000000000000000 ) ) ;
#81824=DIRECTION ( 'NONE',  ( 0.000000000000000000, -0.000000000000000000, 1.000000000000000000 ) ) ;
#81825=CARTESIAN_POINT ( 'NONE',  ( 9.149999999999918643, 2.500000000000000000, 2.165063509461097713 ) ) ;
#81826=FACE_OUTER_BOUND ( 'NONE', #63932, .T. ) ;
#81827=CIRCLE ( 'NONE', #111053, 0.09999999999999982514 ) ;
#81828=CIRCLE ( 'NONE', #25383, 0.06509327318403745899 ) ;
#81829=CARTESIAN_POINT ( 'NONE',  ( 8.949999999999915801, 2.500000000000000000, -1.718653347947326049 ) ) ;
#81830=LINE ( 'NONE', #43229, #100872 ) ;
#81831=FACE_OUTER_BOUND ( 'NONE', #98957, .T. ) ;
#81832=DIRECTION ( 'NONE',  ( -0.000000000000000000, 1.000000000000000000, -0.000000000000000000 ) ) ;
#81833=DIRECTION ( 'NONE',  ( 0.000000000000000000, 0.000000000000000000, 1.000000000000000000 ) ) ;
#81834=ORIENTED_EDGE ( 'NONE', *, *, #8308, .T. ) ;
#81835=CARTESIAN_POINT ( 'NONE',  ( -5.400000000000019895, 12.50000000000000000, 3.637306695894644726 ) ) ;
#81836=ORIENTED_EDGE ( 'NONE', *, *, #4156, .F. ) ;
#81837=ORIENTED_EDGE ( 'NONE', *, *, #94342, .T. ) ;
#81838=DIRECTION ( 'NONE',  ( -0.000000000000000000, 1.000000000000000000, -0.000000000000000000 ) ) ;
#81839=DIRECTION ( 'NONE',  ( 0.000000000000000000, 0.000000000000000000, -1.000000000000000000 ) ) ;
#81840=FACE_OUTER_BOUND ( 'NONE', #41676, .T. ) ;
#81841=DIRECTION ( 'NONE',  ( 0.000000000000000000, 0.000000000000000000, 1.000000000000000000 ) ) ;
#81842=EDGE_CURVE ( 'NONE', #102321, #65003, #13906, .T. ) ;
#81843=DIRECTION ( 'NONE',  ( -0.000000000000000000, -1.000000000000000000, -0.000000000000000000 ) ) ;
#81844=DIRECTION ( 'NONE',  ( -4.274815082592931898E-19, -0.9999939076577903929, -0.003490651415223739937 ) ) ;
#81845=AXIS2_PLACEMENT_3D ( 'NONE', #98177, #78568, #118460 ) ;
#81846=FACE_OUTER_BOUND ( 'NONE', #5737, .T. ) ;
#81847=ORIENTED_EDGE ( 'NONE', *, *, #113606, .F. ) ;
#81848=CONICAL_SURFACE ( 'NONE', #125751, 0.1000000000000000472, 0.003490658503988666988 ) ;
#81849=CONICAL_SURFACE ( 'NONE', #10820, 0.09999999999999982514, 0.003490658503988666988 ) ;
#81850=ORIENTED_EDGE ( 'NONE', *, *, #85649, .F. ) ;
#81851=CIRCLE ( 'NONE', #125757, 0.09999999999999999167 ) ;
#81852=VERTEX_POINT ( 'NONE', #125166 ) ;
#81853=AXIS2_PLACEMENT_3D ( 'NONE', #18063, #37083, #29208 ) ;
#81854=ORIENTED_EDGE ( 'NONE', *, *, #2436, .F. ) ;
#81855=AXIS2_PLACEMENT_3D ( 'NONE', #8231, #57998, #29190 ) ;
#81856=EDGE_CURVE ( 'NONE', #108534, #38221, #30387, .T. ) ;
#81857=VERTEX_POINT ( 'NONE', #65593 ) ;
#81858=CARTESIAN_POINT ( 'NONE',  ( 5.799999999999934985, 2.500000000000000000, -4.230127018922201998 ) ) ;
#81859=CARTESIAN_POINT ( 'NONE',  ( 1.899999999999949507, 2.500000000000000000, 4.083716857408421497 ) ) ;
#81860=CONICAL_SURFACE ( 'NONE', #98577, 0.09999999999999982514, 0.003490658503988666988 ) ;
#81862=DIRECTION ( 'NONE',  ( -0.000000000000000000, 1.000000000000000000, -0.000000000000000000 ) ) ;
#81863=CARTESIAN_POINT ( 'NONE',  ( 87.50000000000001421, -3.413194297214857897, 6.711110875543779386 ) ) ;
#81864=ORIENTED_EDGE ( 'NONE', *, *, #15109, .F. ) ;
#81865=DIRECTION ( 'NONE',  ( 0.000000000000000000, 0.000000000000000000, 1.000000000000000000 ) ) ;
#81866=DIRECTION ( 'NONE',  ( 0.000000000000000000, 1.000000000000000000, 0.000000000000000000 ) ) ;
#81867=DIRECTION ( 'NONE',  ( -0.000000000000000000, 1.000000000000000000, -0.000000000000000000 ) ) ;
#81868=DIRECTION ( 'NONE',  ( 0.000000000000000000, 0.000000000000000000, 1.000000000000000000 ) ) ;
#81869=FACE_OUTER_BOUND ( 'NONE', #31149, .T. ) ;
#81870=VERTEX_POINT ( 'NONE', #72845 ) ;
#81871=ORIENTED_EDGE ( 'NONE', *, *, #49014, .T. ) ;
#81872=VERTEX_POINT ( 'NONE', #104234 ) ;
#81873=DIRECTION ( 'NONE',  ( 0.000000000000000000, 1.000000000000000000, 0.000000000000000000 ) ) ;
#81874=ORIENTED_EDGE ( 'NONE', *, *, #93620, .F. ) ;
#81875=LINE ( 'NONE', #14423, #76013 ) ;
#81877=VECTOR ( 'NONE', #106802, 1000.000000000000000 ) ;
#81878=ADVANCED_FACE ( 'NONE', ( #44677 ), #114686, .T. ) ;
#81879=ORIENTED_EDGE ( 'NONE', *, *, #25569, .F. ) ;
#81880=DIRECTION ( 'NONE',  ( 0.000000000000000000, 0.000000000000000000, 1.000000000000000000 ) ) ;
#81881=CARTESIAN_POINT ( 'NONE',  ( -1.850000000000033396, 2.500000000000000000, -1.818653347947325916 ) ) ;
#81882=DIRECTION ( 'NONE',  ( 0.000000000000000000, 0.000000000000000000, 1.000000000000000000 ) ) ;
#81883=DIRECTION ( 'NONE',  ( -0.000000000000000000, 1.000000000000000000, -0.000000000000000000 ) ) ;
#81884=AXIS2_PLACEMENT_3D ( 'NONE', #23474, #90929, #42489 ) ;
#81886=AXIS2_PLACEMENT_3D ( 'NONE', #127497, #47647, #78408 ) ;
#81887=CARTESIAN_POINT ( 'NONE',  ( 9.349999999999916156, 2.500000000000000000, -1.818653347947326138 ) ) ;
#81888=CIRCLE ( 'NONE', #90207, 0.09999999999999982514 ) ;
#81889=VERTEX_POINT ( 'NONE', #34223 ) ;
#81890=EDGE_CURVE ( 'NONE', #32820, #36161, #124452, .T. ) ;
#81891=EDGE_CURVE ( 'NONE', #101973, #102305, #53454, .T. ) ;
#81893=EDGE_LOOP ( 'NONE', ( #121347, #86922, #60377, #23270 ) ) ;
#81894=ADVANCED_FACE ( 'NONE', ( #114061 ), #111935, .T. ) ;
#81895=CARTESIAN_POINT ( 'NONE',  ( 2.099999999999949463, 2.500000000000000000, 0.6928203230275494784 ) ) ;
#81896=ADVANCED_FACE ( 'NONE', ( #83933 ), #24105, .T. ) ;
#81897=EDGE_CURVE ( 'NONE', #88124, #18723, #40858, .T. ) ;
#81898=CARTESIAN_POINT ( 'NONE',  ( 5.649999999999932854, 12.50000000000000000, 1.753560074763284016 ) ) ;
#81899=CARTESIAN_POINT ( 'NONE',  ( -13.94999999999998863, 2.500000000000000000, -1.918653347947324006 ) ) ;
#81900=CIRCLE ( 'NONE', #37998, 0.09999999999999982514 ) ;
#81901=CIRCLE ( 'NONE', #56753, 0.09999999999999982514 ) ;
#81902=CARTESIAN_POINT ( 'NONE',  ( 4.799999999999937650, 2.500000000000000000, -3.983716857408426293 ) ) ;
#81903=EDGE_LOOP ( 'NONE', ( #12688, #36063, #116971, #12265 ) ) ;
#81904=AXIS2_PLACEMENT_3D ( 'NONE', #37523, #77430, #8034 ) ;
#81905=VECTOR ( 'NONE', #52547, 1000.000000000000000 ) ;
#81906=CIRCLE ( 'NONE', #111147, 0.06509327318403745899 ) ;
#81907=ORIENTED_EDGE ( 'NONE', *, *, #40358, .T. ) ;
#81908=DIRECTION ( 'NONE',  ( -4.274815082592931898E-19, -0.9999939076577903929, -0.003490651415223739937 ) ) ;
#81909=DIRECTION ( 'NONE',  ( 0.000000000000000000, 0.000000000000000000, 1.000000000000000000 ) ) ;
#81910=ADVANCED_FACE ( 'NONE', ( #108088 ), #74285, .T. ) ;
#81911=CIRCLE ( 'NONE', #44257, 0.1000000000000002554 ) ;
#81912=DIRECTION ( 'NONE',  ( 0.000000000000000000, 0.000000000000000000, 1.000000000000000000 ) ) ;
#81913=CARTESIAN_POINT ( 'NONE',  ( -3.750000000000025757, 12.50000000000000000, -2.792790559304616504 ) ) ;
#81914=EDGE_LOOP ( 'NONE', ( #79464, #23543, #117508, #61173 ) ) ;
#81915=EDGE_CURVE ( 'NONE', #84545, #2147, #93167, .T. ) ;
#81917=ADVANCED_FACE ( 'NONE', ( #18430 ), #125784, .T. ) ;
#81918=DIRECTION ( 'NONE',  ( 0.000000000000000000, 1.000000000000000000, 0.000000000000000000 ) ) ;
#81919=EDGE_LOOP ( 'NONE', ( #92208, #22941 ) ) ;
#81920=CARTESIAN_POINT ( 'NONE',  ( 10.84999999999991260, 12.50000000000000000, -2.230156782645139391 ) ) ;
#81921=ORIENTED_EDGE ( 'NONE', *, *, #107038, .F. ) ;
#81922=DIRECTION ( 'NONE',  ( 0.000000000000000000, 0.000000000000000000, 1.000000000000000000 ) ) ;
#81923=ORIENTED_EDGE ( 'NONE', *, *, #121835, .F. ) ;
#81925=LINE ( 'NONE', #91116, #25027 ) ;
#81926=VERTEX_POINT ( 'NONE', #86514 ) ;
#81927=ORIENTED_EDGE ( 'NONE', *, *, #90955, .T. ) ;
#81928=DIRECTION ( 'NONE',  ( -4.274815082592931898E-19, -0.9999939076577903929, -0.003490651415223739937 ) ) ;
#81929=CARTESIAN_POINT ( 'NONE',  ( -4.150000000000025224, 2.500000000000000000, 6.595190528383296780 ) ) ;
#81930=CARTESIAN_POINT ( 'NONE',  ( 6.849999999999927702, 2.500000000000000000, 1.818653347947321475 ) ) ;
#81933=AXIS2_PLACEMENT_3D ( 'NONE', #124761, #23323, #62633 ) ;
#81934=CARTESIAN_POINT ( 'NONE',  ( 0.5999999999999612310, 12.50000000000000000, -0.4115034346978134749 ) ) ;
#81935=CARTESIAN_POINT ( 'NONE',  ( 2.099999999999950351, 2.500000000000000000, -4.922947341949753586 ) ) ;
#81936=CIRCLE ( 'NONE', #40197, 0.1000000000000002554 ) ;
#81937=AXIS2_PLACEMENT_3D ( 'NONE', #127732, #78656, #129053 ) ;
#81938=ADVANCED_FACE ( 'NONE', ( #97633 ), #98269, .T. ) ;
#81939=CARTESIAN_POINT ( 'NONE',  ( 14.14999999999989733, 2.500000000000000000, 2.857883832488649301 ) ) ;
#81940=DIRECTION ( 'NONE',  ( 0.000000000000000000, 0.000000000000000000, -1.000000000000000000 ) ) ;
#81941=CONICAL_SURFACE ( 'NONE', #35996, 0.1000000000000002554, 0.003490658503988666988 ) ;
#81942=AXIS2_PLACEMENT_3D ( 'NONE', #91701, #23597, #3317 ) ;
#81943=ORIENTED_EDGE ( 'NONE', *, *, #9965, .T. ) ;
#81944=ADVANCED_FACE ( 'NONE', ( #7956 ), #78506, .T. ) ;
#81945=VECTOR ( 'NONE', #73609, 1000.000000000000000 ) ;
#81946=EDGE_LOOP ( 'NONE', ( #9761, #32358, #110385, #37521 ) ) ;
#81947=CARTESIAN_POINT ( 'NONE',  ( -10.84999999999999964, 2.500000000000000000, 5.802370205355744659 ) ) ;
#81948=ORIENTED_EDGE ( 'NONE', *, *, #3443, .F. ) ;
#81949=CARTESIAN_POINT ( 'NONE',  ( -6.650000000000014566, 2.500000000000000000, 5.802370205355744659 ) ) ;
#81950=CARTESIAN_POINT ( 'NONE',  ( 6.649999999999929301, 2.500000000000000000, -2.265063509461101798 ) ) ;
#81951=AXIS2_PLACEMENT_3D ( 'NONE', #107583, #38206, #78785 ) ;
#81952=DIRECTION ( 'NONE',  ( 0.000000000000000000, 1.000000000000000000, 0.000000000000000000 ) ) ;
#81953=CONICAL_SURFACE ( 'NONE', #58991, 0.09999999999999982514, 0.003490658503988666988 ) ;
#81954=ORIENTED_EDGE ( 'NONE', *, *, #69191, .T. ) ;
#81955=ORIENTED_EDGE ( 'NONE', *, *, #25960, .T. ) ;
#81956=FACE_BOUND ( 'NONE', #38794, .T. ) ;
#81957=ORIENTED_EDGE ( 'NONE', *, *, #120492, .T. ) ;
#81958=ADVANCED_FACE ( 'NONE', ( #17774 ), #26258, .T. ) ;
#81959=DIRECTION ( 'NONE',  ( -0.000000000000000000, 1.000000000000000000, -0.000000000000000000 ) ) ;
#81960=DIRECTION ( 'NONE',  ( 0.000000000000000000, -0.000000000000000000, 1.000000000000000000 ) ) ;
#81961=EDGE_CURVE ( 'NONE', #101480, #86613, #45973, .T. ) ;
#81962=PLANE ( 'NONE',  #7467 ) ;
#81963=DIRECTION ( 'NONE',  ( 0.000000000000000000, 0.000000000000000000, 1.000000000000000000 ) ) ;
#81964=DIRECTION ( 'NONE',  ( 0.000000000000000000, 0.000000000000000000, 1.000000000000000000 ) ) ;
#81965=EDGE_CURVE ( 'NONE', #103567, #84006, #51317, .T. ) ;
#81966=CARTESIAN_POINT ( 'NONE',  ( 5.199999999999933564, 12.50000000000000000, 0.2813168883297361700 ) ) ;
#81967=FACE_OUTER_BOUND ( 'NONE', #105118, .T. ) ;
#81968=DIRECTION ( 'NONE',  ( 0.000000000000000000, 1.000000000000000000, 0.000000000000000000 ) ) ;
#81969=CARTESIAN_POINT ( 'NONE',  ( 5.649999999999932854, 2.500000000000000000, 1.818653347947321475 ) ) ;
#81970=DIRECTION ( 'NONE',  ( -0.000000000000000000, 1.000000000000000000, -0.000000000000000000 ) ) ;
#81971=DIRECTION ( 'NONE',  ( 0.000000000000000000, -0.000000000000000000, 1.000000000000000000 ) ) ;
#81972=EDGE_CURVE ( 'NONE', #38064, #83506, #115983, .T. ) ;
#81973=VERTEX_POINT ( 'NONE', #56413 ) ;
#81974=EDGE_LOOP ( 'NONE', ( #42485, #116549 ) ) ;
#81975=ORIENTED_EDGE ( 'NONE', *, *, #88403, .T. ) ;
#81976=CARTESIAN_POINT ( 'NONE',  ( 6.849999999999927702, 2.500000000000000000, 2.511473670974873507 ) ) ;
#81977=ORIENTED_EDGE ( 'NONE', *, *, #85769, .F. ) ;
#81978=DIRECTION ( 'NONE',  ( -4.274815082592931898E-19, -0.9999939076577903929, -0.003490651415223739937 ) ) ;
#81979=CARTESIAN_POINT ( 'NONE',  ( -2.100000000000033840, 2.500000000000000000, 3.637306695894644726 ) ) ;
#81980=ORIENTED_EDGE ( 'NONE', *, *, #50281, .T. ) ;
#81981=ORIENTED_EDGE ( 'NONE', *, *, #105638, .F. ) ;
#81982=ORIENTED_EDGE ( 'NONE', *, *, #72016, .F. ) ;
#81983=DIRECTION ( 'NONE',  ( 0.000000000000000000, 0.000000000000000000, 1.000000000000000000 ) ) ;
#81984=CIRCLE ( 'NONE', #54784, 0.06509327318403745899 ) ;
#81985=PLANE ( 'NONE',  #117811 ) ;
#81986=( NAMED_UNIT ( * ) PLANE_ANGLE_UNIT ( ) SI_UNIT ( $, .RADIAN. ) );
#81987=DIRECTION ( 'NONE',  ( -0.000000000000000000, 1.000000000000000000, -0.000000000000000000 ) ) ;
#81988=DIRECTION ( 'NONE',  ( -0.000000000000000000, -1.000000000000000000, -0.000000000000000000 ) ) ;
#81989=FACE_OUTER_BOUND ( 'NONE', #59707, .T. ) ;
#81990=CARTESIAN_POINT ( 'NONE',  ( 2.949999999999945111, 12.50000000000000000, 2.165063509461097713 ) ) ;
#81991=EDGE_CURVE ( 'NONE', #54491, #37534, #68011, .T. ) ;
#81992=ORIENTED_EDGE ( 'NONE', *, *, #89306, .T. ) ;
#81994=CIRCLE ( 'NONE', #2553, 0.06509327318403745899 ) ;
#81995=CARTESIAN_POINT ( 'NONE',  ( 13.34999999999990017, 2.500000000000000000, 1.372243186433545370 ) ) ;
#81996=VERTEX_POINT ( 'NONE', #36798 ) ;
#81997=CONICAL_SURFACE ( 'NONE', #79844, 0.09999999999999982514, 0.003490658503988666988 ) ;
#81998=ORIENTED_EDGE ( 'NONE', *, *, #4228, .F. ) ;
#81999=AXIS2_PLACEMENT_3D ( 'NONE', #124709, #32490, #82209 ) ;
#82000=EDGE_LOOP ( 'NONE', ( #103009, #37412 ) ) ;
#82001=DIRECTION ( 'NONE',  ( 0.000000000000000000, 0.000000000000000000, 1.000000000000000000 ) ) ;
#82002=ORIENTED_EDGE ( 'NONE', *, *, #38205, .T. ) ;
#82003=EDGE_LOOP ( 'NONE', ( #16963, #7159, #18860, #42979 ) ) ;
#82004=ORIENTED_EDGE ( 'NONE', *, *, #53414, .T. ) ;
#82005=AXIS2_PLACEMENT_3D ( 'NONE', #106067, #115206, #106697 ) ;
#82006=CARTESIAN_POINT ( 'NONE',  ( -7.900000000000014566, 12.50000000000000000, -5.088040615133791356 ) ) ;
#82007=CIRCLE ( 'NONE', #125907, 0.09999999999999982514 ) ;
#82008=FACE_OUTER_BOUND ( 'NONE', #38321, .T. ) ;
#82009=ADVANCED_FACE ( 'NONE', ( #7302 ), #11576, .T. ) ;
#82010=DIRECTION ( 'NONE',  ( 0.000000000000000000, 0.000000000000000000, 1.000000000000000000 ) ) ;
#82011=VECTOR ( 'NONE', #105351, 1000.000000000000000 ) ;
#82012=CARTESIAN_POINT ( 'NONE',  ( -5.000000000000022204, 12.50000000000000000, -0.7579135962115916003 ) ) ;
#82013=CARTESIAN_POINT ( 'NONE',  ( -1.250000000000037526, 2.500000000000000000, -5.902370205355750521 ) ) ;
#82014=AXIS2_PLACEMENT_3D ( 'NONE', #83396, #117818, #47823 ) ;
#82015=DIRECTION ( 'NONE',  ( 0.000000000000000000, 1.000000000000000000, 0.000000000000000000 ) ) ;
#82016=EDGE_LOOP ( 'NONE', ( #129235, #84950 ) ) ;
#82017=CARTESIAN_POINT ( 'NONE',  ( 4.799999999999939426, 12.50000000000000000, -4.676537180435977881 ) ) ;
#82018=ORIENTED_EDGE ( 'NONE', *, *, #20352, .T. ) ;
#82019=DIRECTION ( 'NONE',  ( 0.000000000000000000, 1.000000000000000000, 0.000000000000000000 ) ) ;
#82020=ORIENTED_EDGE ( 'NONE', *, *, #113933, .T. ) ;
#82021=DIRECTION ( 'NONE',  ( 0.000000000000000000, 1.000000000000000000, 0.000000000000000000 ) ) ;
#82022=ADVANCED_FACE ( 'NONE', ( #88444 ), #45048, .T. ) ;
#82023=ORIENTED_EDGE ( 'NONE', *, *, #25295, .F. ) ;
#82025=CARTESIAN_POINT ( 'NONE',  ( 14.79999999999989413, 12.50000000000000000, -0.4115034346978156399 ) ) ;
#82026=ORIENTED_EDGE ( 'NONE', *, *, #22464, .F. ) ;
#82027=EDGE_LOOP ( 'NONE', ( #40085, #25727, #59999, #30479 ) ) ;
#82028=FACE_OUTER_BOUND ( 'NONE', #90058, .T. ) ;
#82029=PLANE ( 'NONE',  #59734 ) ;
#82030=DIRECTION ( 'NONE',  ( 0.000000000000000000, -0.9999939076577903929, 0.003490651415223739937 ) ) ;
#82031=FACE_OUTER_BOUND ( 'NONE', #127681, .T. ) ;
#82032=DIRECTION ( 'NONE',  ( -4.274815082592931898E-19, -0.9999939076577903929, -0.003490651415223739937 ) ) ;
#82033=ORIENTED_EDGE ( 'NONE', *, *, #23540, .F. ) ;
#82034=CARTESIAN_POINT ( 'NONE',  ( 2.500000000000002220, -1.500000000000000000, 10.00000000000000178 ) ) ;
#82035=VECTOR ( 'NONE', #1317, 1000.000000000000000 ) ;
#82036=CONICAL_SURFACE ( 'NONE', #102968, 0.1000000000000002554, 0.003490658503988666988 ) ;
#82037=ORIENTED_EDGE ( 'NONE', *, *, #70845, .F. ) ;
#82038=DIRECTION ( 'NONE',  ( 0.000000000000000000, -0.000000000000000000, 1.000000000000000000 ) ) ;
#82039=DIRECTION ( 'NONE',  ( 0.000000000000000000, 0.000000000000000000, 1.000000000000000000 ) ) ;
#82040=AXIS2_PLACEMENT_3D ( 'NONE', #15671, #103435, #115822 ) ;
#82041=AXIS2_PLACEMENT_3D ( 'NONE', #57426, #124233, #45038 ) ;
#82042=VECTOR ( 'NONE', #14036, 1000.000000000000000 ) ;
#82043=ADVANCED_FACE ( 'NONE', ( #118555 ), #20000, .T. ) ;
#82044=CIRCLE ( 'NONE', #59075, 0.06509327318403745899 ) ;
#82045=CIRCLE ( 'NONE', #466, 0.09999999999999982514 ) ;
#82047=LINE ( 'NONE', #61790, #128410 ) ;
#82048=DIRECTION ( 'NONE',  ( -4.274815082592931898E-19, -0.9999939076577903929, -0.003490651415223739937 ) ) ;
#82049=CARTESIAN_POINT ( 'NONE',  ( -5.400000000000020783, 12.50000000000000000, 0.6277270498435120194 ) ) ;
#82050=FACE_OUTER_BOUND ( 'NONE', #102649, .T. ) ;
#82051=ORIENTED_EDGE ( 'NONE', *, *, #20204, .T. ) ;
#82052=AXIS2_PLACEMENT_3D ( 'NONE', #90066, #393, #69139 ) ;
#82053=ADVANCED_FACE ( 'NONE', ( #68816 ), #107532, .T. ) ;
#82054=CARTESIAN_POINT ( 'NONE',  ( -11.25000000000000178, 12.50000000000000000, -5.802370205355746435 ) ) ;
#82055=CARTESIAN_POINT ( 'NONE',  ( -4.999999999999986677, 12.50000000000000000, 4.330127018922196314 ) ) ;
#82056=CARTESIAN_POINT ( 'NONE',  ( 3.099999999999945022, 12.50000000000000000, -4.676537180435978769 ) ) ;
#82057=ORIENTED_EDGE ( 'NONE', *, *, #125513, .F. ) ;
#82058=ADVANCED_FACE ( 'NONE', ( #66231 ), #74086, .T. ) ;
#82059=EDGE_CURVE ( 'NONE', #31935, #53009, #128479, .T. ) ;
#82061=EDGE_CURVE ( 'NONE', #83059, #127177, #39391, .T. ) ;
#82063=DIRECTION ( 'NONE',  ( 0.000000000000000000, 0.000000000000000000, -1.000000000000000000 ) ) ;
#82064=VECTOR ( 'NONE', #65799, 1000.000000000000000 ) ;
#82065=EDGE_LOOP ( 'NONE', ( #14157, #20130 ) ) ;
#82066=ORIENTED_EDGE ( 'NONE', *, *, #34924, .T. ) ;
#82067=DIRECTION ( 'NONE',  ( -0.000000000000000000, -1.000000000000000000, -0.000000000000000000 ) ) ;
#82068=EDGE_CURVE ( 'NONE', #87872, #64350, #121139, .T. ) ;
#82069=EDGE_CURVE ( 'NONE', #93103, #50389, #99583, .T. ) ;
#82070=ORIENTED_EDGE ( 'NONE', *, *, #80598, .T. ) ;
#82071=CARTESIAN_POINT ( 'NONE',  ( 16.72050902516516757, -2.552201582241029332, -5.918448581785260565 ) ) ;
#82072=PLANE ( 'NONE',  #2727 ) ;
#82073=EDGE_CURVE ( 'NONE', #112141, #126712, #28118, .T. ) ;
#82074=CARTESIAN_POINT ( 'NONE',  ( 16.09541403888798783, 2.463474929527698531, 3.723514363710399344 ) ) ;
#82075=AXIS2_PLACEMENT_3D ( 'NONE', #87986, #25870, #17972 ) ;
#82076=ORIENTED_EDGE ( 'NONE', *, *, #113564, .T. ) ;
#82077=AXIS2_PLACEMENT_3D ( 'NONE', #103838, #4310, #66475 ) ;
#82078=EDGE_CURVE ( 'NONE', #103138, #1435, #86588, .T. ) ;
#82079=AXIS2_PLACEMENT_3D ( 'NONE', #73414, #121238, #4026 ) ;
#82081=EDGE_CURVE ( 'NONE', #68676, #61297, #120058, .T. ) ;
#82082=CARTESIAN_POINT ( 'NONE',  ( -2.100000000000033396, 12.50000000000000000, 0.6928203230275494784 ) ) ;
#82083=AXIS2_PLACEMENT_3D ( 'NONE', #123761, #33485, #74038 ) ;
#82084=ADVANCED_FACE ( 'NONE', ( #110668 ), #7170, .T. ) ;
#82085=ORIENTED_EDGE ( 'NONE', *, *, #84386, .T. ) ;
#82086=CONICAL_SURFACE ( 'NONE', #61162, 0.09999999999999982514, 0.003490658503988666988 ) ;
#82088=ORIENTED_EDGE ( 'NONE', *, *, #9385, .T. ) ;
#82089=ORIENTED_EDGE ( 'NONE', *, *, #38031, .T. ) ;
#82090=CARTESIAN_POINT ( 'NONE',  ( -3.350000000000031619, 12.50000000000000000, -7.122917578226816815 ) ) ;
#82091=CARTESIAN_POINT ( 'NONE',  ( -4.400000000000025224, 2.500000000000000000, 0.3464101615137735735 ) ) ;
#82093=FACE_BOUND ( 'NONE', #56815, .T. ) ;
#82094=VERTEX_POINT ( 'NONE', #20369 ) ;
#82095=CARTESIAN_POINT ( 'NONE',  ( -0.6500000000000398792, 12.50000000000000000, -2.511473670974877948 ) ) ;
#82096=DIRECTION ( 'NONE',  ( 0.000000000000000000, 0.000000000000000000, -1.000000000000000000 ) ) ;
#82097=CIRCLE ( 'NONE', #67393, 0.09999999999999982514 ) ;
#82098=EDGE_LOOP ( 'NONE', ( #103742, #43075, #15976, #14635 ) ) ;
#82099=AXIS2_PLACEMENT_3D ( 'NONE', #121065, #9822, #60857 ) ;
#82100=CARTESIAN_POINT ( 'NONE',  ( 8.549999999999918998, 12.50000000000000000, 6.776507416713035248 ) ) ;
#82101=DIRECTION ( 'NONE',  ( 0.000000000000000000, 0.000000000000000000, 1.000000000000000000 ) ) ;
#82102=VECTOR ( 'NONE', #90197, 1000.000000000000000 ) ;
#82103=CONICAL_SURFACE ( 'NONE', #19397, 0.1000000000000002554, 0.003490658503988666988 ) ;
#82104=AXIS2_PLACEMENT_3D ( 'NONE', #98233, #89707, #33 ) ;
#82105=DIRECTION ( 'NONE',  ( 0.000000000000000000, -0.000000000000000000, 1.000000000000000000 ) ) ;
#82106=CARTESIAN_POINT ( 'NONE',  ( 10.19999999999991225, 12.50000000000000000, 4.048810130592458201 ) ) ;
#82108=PLANE ( 'NONE',  #63949 ) ;
#82109=AXIS2_PLACEMENT_3D ( 'NONE', #13671, #1920, #43169 ) ;
#82110=DIRECTION ( 'NONE',  ( 0.000000000000000000, 0.000000000000000000, 1.000000000000000000 ) ) ;
#82112=AXIS2_PLACEMENT_3D ( 'NONE', #22748, #32571, #50261 ) ;
#82113=ORIENTED_EDGE ( 'NONE', *, *, #89257, .F. ) ;
#82114=ORIENTED_EDGE ( 'NONE', *, *, #94428, .F. ) ;
#82115=EDGE_LOOP ( 'NONE', ( #12609, #43319 ) ) ;
#82116=LINE ( 'NONE', #12080, #3549 ) ;
#82117=CARTESIAN_POINT ( 'NONE',  ( 3.749999999999938716, 2.500000000000000000, 7.288010851410849256 ) ) ;
#82118=LINE ( 'NONE', #111578, #29985 ) ;
#82119=ORIENTED_EDGE ( 'NONE', *, *, #83446, .T. ) ;
#82120=FACE_BOUND ( 'NONE', #41391, .T. ) ;
#82121=FACE_OUTER_BOUND ( 'NONE', #110250, .T. ) ;
#82122=DIRECTION ( 'NONE',  ( 0.000000000000000000, -0.9999939076577903929, 0.003490651415223739937 ) ) ;
#82123=EDGE_CURVE ( 'NONE', #19888, #74443, #78307, .T. ) ;
#82125=CARTESIAN_POINT ( 'NONE',  ( -0.2000000000000399791, 12.50000000000000000, -4.611443907251939756 ) ) ;
#82126=EDGE_CURVE ( 'NONE', #51796, #47551, #60926, .T. ) ;
#82127=CARTESIAN_POINT ( 'NONE',  ( -9.550000000000006040, 2.500000000000000000, 2.065063509461097624 ) ) ;
#82128=CARTESIAN_POINT ( 'NONE',  ( 6.849999999999927702, 12.50000000000000000, 1.883746621131358934 ) ) ;
#82129=CARTESIAN_POINT ( 'NONE',  ( 11.44999999999990514, 2.500000000000000000, 2.411473670974873862 ) ) ;
#82130=LINE ( 'NONE', #72961, #9474 ) ;
#82131=CONICAL_SURFACE ( 'NONE', #54926, 0.09999999999999982514, 0.003490658503988666988 ) ;
#82132=CONICAL_SURFACE ( 'NONE', #65392, 0.09999999999999982514, 0.003490658503988666988 ) ;
#82133=DIRECTION ( 'NONE',  ( -4.274815082592931898E-19, -0.9999939076577903929, -0.003490651415223739937 ) ) ;
#82134=EDGE_CURVE ( 'NONE', #49056, #107837, #120352, .T. ) ;
#82136=AXIS2_PLACEMENT_3D ( 'NONE', #93497, #86226, #44385 ) ;
#82137=EDGE_CURVE ( 'NONE', #64505, #39552, #36452, .T. ) ;
#82138=ORIENTED_EDGE ( 'NONE', *, *, #81406, .F. ) ;
#82139=ORIENTED_EDGE ( 'NONE', *, *, #97756, .F. ) ;
#82140=VERTEX_POINT ( 'NONE', #9900 ) ;
#82141=AXIS2_PLACEMENT_3D ( 'NONE', #83405, #8517, #7226 ) ;
#82142=ORIENTED_EDGE ( 'NONE', *, *, #67280, .F. ) ;
#82143=VERTEX_POINT ( 'NONE', #22320 ) ;
#82144=AXIS2_PLACEMENT_3D ( 'NONE', #116789, #109567, #58545 ) ;
#82146=ORIENTED_EDGE ( 'NONE', *, *, #35540, .F. ) ;
#82147=ORIENTED_EDGE ( 'NONE', *, *, #38257, .T. ) ;
#82148=CIRCLE ( 'NONE', #69618, 0.06509327318403745899 ) ;
#82149=AXIS2_PLACEMENT_3D ( 'NONE', #41671, #81568, #3016 ) ;
#82150=AXIS2_PLACEMENT_3D ( 'NONE', #4258, #92021, #2326 ) ;
#82151=DIRECTION ( 'NONE',  ( 0.000000000000000000, 0.000000000000000000, 1.000000000000000000 ) ) ;
#82152=LINE ( 'NONE', #81511, #33010 ) ;
#82153=DIRECTION ( 'NONE',  ( 0.000000000000000000, 0.000000000000000000, -1.000000000000000000 ) ) ;
#82154=CARTESIAN_POINT ( 'NONE',  ( 12.69999999999990159, 2.500000000000000000, 4.576537180435972019 ) ) ;
#82155=CONICAL_SURFACE ( 'NONE', #8969, 0.1000000000000002554, 0.003490658503988666988 ) ;
#82156=AXIS2_PLACEMENT_3D ( 'NONE', #22784, #103263, #81678 ) ;
#82157=EDGE_LOOP ( 'NONE', ( #120567, #119256 ) ) ;
#82158=LINE ( 'NONE', #61229, #119514 ) ;
#82159=CIRCLE ( 'NONE', #128232, 0.06509327318403745899 ) ;
#82160=ORIENTED_EDGE ( 'NONE', *, *, #79204, .F. ) ;
#82161=ORIENTED_EDGE ( 'NONE', *, *, #55346, .T. ) ;
#82162=DIRECTION ( 'NONE',  ( 0.000000000000000000, 1.000000000000000000, 0.000000000000000000 ) ) ;
#82163=CARTESIAN_POINT ( 'NONE',  ( 6.249999999999932498, 2.500000000000000000, 5.702370205355745014 ) ) ;
#82164=VERTEX_POINT ( 'NONE', #98921 ) ;
#82165=EDGE_LOOP ( 'NONE', ( #96717, #46126, #34232, #13738 ) ) ;
#82166=AXIS2_PLACEMENT_3D ( 'NONE', #72906, #64993, #44744 ) ;
#82167=ADVANCED_FACE ( 'NONE', ( #11823 ), #68, .T. ) ;
#82168=CARTESIAN_POINT ( 'NONE',  ( 10.64999999999991331, 2.500000000000000000, 6.148780366869520897 ) ) ;
#82169=DIRECTION ( 'NONE',  ( 0.000000000000000000, -0.9999939076577903929, 0.003490651415223739937 ) ) ;
#82170=FACE_OUTER_BOUND ( 'NONE', #6137, .T. ) ;
#82171=CARTESIAN_POINT ( 'NONE',  ( 13.34999999999989662, 2.500000000000000000, -1.472243186433550122 ) ) ;
#82172=LINE ( 'NONE', #21307, #108760 ) ;
#82173=CIRCLE ( 'NONE', #34060, 0.06509327318403745899 ) ;
#82174=EDGE_LOOP ( 'NONE', ( #19241, #97779, #7616, #64856 ) ) ;
#82175=LINE ( 'NONE', #122109, #46919 ) ;
#82176=VECTOR ( 'NONE', #44772, 1000.000000000000000 ) ;
#82178=ORIENTED_EDGE ( 'NONE', *, *, #63753, .F. ) ;
#82179=CARTESIAN_POINT ( 'NONE',  ( 17.50000000000000000, 2.499999999999999556, 2.666666666666668739 ) ) ;
#82180=DIRECTION ( 'NONE',  ( 0.000000000000000000, 0.000000000000000000, -1.000000000000000000 ) ) ;
#82181=DIRECTION ( 'NONE',  ( -0.000000000000000000, 1.000000000000000000, -0.000000000000000000 ) ) ;
#82182=EDGE_CURVE ( 'NONE', #13197, #6403, #49204, .T. ) ;
#82183=CARTESIAN_POINT ( 'NONE',  ( -7.500000000000013323, 2.500000000000000000, 5.022947341949748790 ) ) ;
#82184=EDGE_CURVE ( 'NONE', #65087, #43418, #90805, .T. ) ;
#82185=FACE_OUTER_BOUND ( 'NONE', #125771, .T. ) ;
#82186=CIRCLE ( 'NONE', #36127, 0.06509327318403745899 ) ;
#82187=VERTEX_POINT ( 'NONE', #129054 ) ;
#82188=CIRCLE ( 'NONE', #88519, 0.09999999999999982514 ) ;
#82189=CONICAL_SURFACE ( 'NONE', #94797, 0.1000000000000002554, 0.003490658503988666988 ) ;
#82190=CARTESIAN_POINT ( 'NONE',  ( 5.649999999999934630, 12.50000000000000000, 6.841600689897072485 ) ) ;
#82191=CONICAL_SURFACE ( 'NONE', #98908, 0.1000000000000002554, 0.003490658503988666988 ) ;
#82192=CARTESIAN_POINT ( 'NONE',  ( -11.84999999999999787, 2.500000000000000000, -2.611473670974873595 ) ) ;
#82193=ORIENTED_EDGE ( 'NONE', *, *, #17803, .T. ) ;
#82194=EDGE_LOOP ( 'NONE', ( #60484, #19439 ) ) ;
#82195=ADVANCED_FACE ( 'NONE', ( #119210 ), #69882, .T. ) ;
#82196=EDGE_LOOP ( 'NONE', ( #129593, #121286, #71676, #4552 ) ) ;
#82197=CARTESIAN_POINT ( 'NONE',  ( 17.50000000000000000, -0.9166666666666678509, 10.00000000000000178 ) ) ;
#82198=FACE_OUTER_BOUND ( 'NONE', #101659, .T. ) ;
#82200=CARTESIAN_POINT ( 'NONE',  ( 9.399999999999915090, 12.50000000000000000, 3.983716857408420964 ) ) ;
#82201=CARTESIAN_POINT ( 'NONE',  ( -6.850000000000017408, 2.500000000000000000, -1.718653347947325827 ) ) ;
#82202=CARTESIAN_POINT ( 'NONE',  ( -12.09999999999999609, 12.50000000000000000, -4.395220292106237103 ) ) ;
#82203=AXIS2_PLACEMENT_3D ( 'NONE', #119409, #78880, #38972 ) ;
#82204=CARTESIAN_POINT ( 'NONE',  ( 2.049999999999948308, 2.500000000000000000, 6.595190528383296780 ) ) ;
#82205=CIRCLE ( 'NONE', #90594, 0.06509327318403745899 ) ;
#82206=AXIS2_PLACEMENT_3D ( 'NONE', #97433, #109844, #119646 ) ;
#82207=CARTESIAN_POINT ( 'NONE',  ( -5.600000000000023626, 12.50000000000000000, -3.918623584224389056 ) ) ;
#82208=CIRCLE ( 'NONE', #71745, 0.06509327318403745899 ) ;
#82209=DIRECTION ( 'NONE',  ( 0.000000000000000000, 0.000000000000000000, 1.000000000000000000 ) ) ;
#82210=AXIS2_PLACEMENT_3D ( 'NONE', #113690, #33211, #53485 ) ;
#82211=ORIENTED_EDGE ( 'NONE', *, *, #101434, .F. ) ;
#82213=CARTESIAN_POINT ( 'NONE',  ( -2.300000000000033573, 2.500000000000000000, 0.3464101615137735735 ) ) ;
#82214=CARTESIAN_POINT ( 'NONE',  ( 11.24999999999990585, 12.50000000000000000, -5.802370205355749988 ) ) ;
#82215=CARTESIAN_POINT ( 'NONE',  ( -8.550000000000014921, 2.500000000000000000, -6.148780366869520897 ) ) ;
#82216=VERTEX_POINT ( 'NONE', #70116 ) ;
#82217=DIRECTION ( 'NONE',  ( 0.000000000000000000, 0.000000000000000000, -1.000000000000000000 ) ) ;
#82218=EDGE_CURVE ( 'NONE', #111323, #111265, #110040, .T. ) ;
#82219=CARTESIAN_POINT ( 'NONE',  ( -1.450000000000035039, 2.500000000000000000, -2.511473670974877948 ) ) ;
#82220=CARTESIAN_POINT ( 'NONE',  ( -13.54999999999998828, 12.50000000000000000, 1.883746621131362931 ) ) ;
#82221=ORIENTED_EDGE ( 'NONE', *, *, #109075, .F. ) ;
#82222=CIRCLE ( 'NONE', #17446, 0.06509327318403743123 ) ;
#82223=VECTOR ( 'NONE', #111911, 1000.000000000000000 ) ;
#82224=EDGE_CURVE ( 'NONE', #65883, #12959, #11382, .T. ) ;
#82225=ADVANCED_FACE ( 'NONE', ( #53690 ), #19713, .T. ) ;
#82226=EDGE_CURVE ( 'NONE', #82230, #106895, #13430, .T. ) ;
#82227=EDGE_LOOP ( 'NONE', ( #61291, #38828 ) ) ;
#82228=CARTESIAN_POINT ( 'NONE',  ( 11.04999999999991189, 2.500000000000000000, 6.148780366869520897 ) ) ;
#82229=AXIS2_PLACEMENT_3D ( 'NONE', #124079, #93983, #124726 ) ;
#82230=VERTEX_POINT ( 'NONE', #94903 ) ;
#82231=VECTOR ( 'NONE', #95474, 1000.000000000000000 ) ;
#82232=ORIENTED_EDGE ( 'NONE', *, *, #2939, .T. ) ;
#82233=DIRECTION ( 'NONE',  ( 0.000000000000000000, 1.000000000000000000, 0.000000000000000000 ) ) ;
#82234=CONICAL_SURFACE ( 'NONE', #86417, 0.1000000000000002554, 0.003490658503988666988 ) ;
#82235=ADVANCED_FACE ( 'NONE', ( #14390 ), #55308, .T. ) ;
#82236=AXIS2_PLACEMENT_3D ( 'NONE', #66249, #45345, #43426 ) ;
#82237=EDGE_CURVE ( 'NONE', #64702, #66161, #112619, .T. ) ;
#82238=DIRECTION ( 'NONE',  ( -0.000000000000000000, -1.000000000000000000, -0.000000000000000000 ) ) ;
#82239=PLANE ( 'NONE',  #14981 ) ;
#82240=DIRECTION ( 'NONE',  ( 0.000000000000000000, 0.000000000000000000, -1.000000000000000000 ) ) ;
#82241=CIRCLE ( 'NONE', #21698, 0.06509327318403745899 ) ;
#82242=ORIENTED_EDGE ( 'NONE', *, *, #36160, .T. ) ;
#82243=VECTOR ( 'NONE', #69589, 1000.000000000000000 ) ;
#82244=AXIS2_PLACEMENT_3D ( 'NONE', #53243, #102338, #2840 ) ;
#82245=EDGE_CURVE ( 'NONE', #98256, #81821, #88754, .T. ) ;
#82246=CARTESIAN_POINT ( 'NONE',  ( -2.900000000000029221, 2.500000000000000000, -5.022947341949754119 ) ) ;
#82247=AXIS2_PLACEMENT_3D ( 'NONE', #75073, #126094, #34523 ) ;
#82248=ORIENTED_EDGE ( 'NONE', *, *, #128652, .F. ) ;
#82249=VECTOR ( 'NONE', #85862, 1000.000000000000000 ) ;
#82250=DIRECTION ( 'NONE',  ( -0.000000000000000000, 1.000000000000000000, -0.000000000000000000 ) ) ;
#82251=EDGE_CURVE ( 'NONE', #24335, #90263, #83165, .T. ) ;
#82252=DIRECTION ( 'NONE',  ( -4.274815082592931898E-19, -0.9999939076577903929, -0.003490651415223739937 ) ) ;
#82253=EDGE_CURVE ( 'NONE', #117879, #77488, #61583, .T. ) ;
#82254=AXIS2_PLACEMENT_3D ( 'NONE', #49859, #31492, #79322 ) ;
#82255=ORIENTED_EDGE ( 'NONE', *, *, #119744, .F. ) ;
#82256=ORIENTED_EDGE ( 'NONE', *, *, #57574, .F. ) ;
#82257=ORIENTED_EDGE ( 'NONE', *, *, #89579, .T. ) ;
#82259=DIRECTION ( 'NONE',  ( 0.000000000000000000, 1.000000000000000000, 0.000000000000000000 ) ) ;
#82260=CARTESIAN_POINT ( 'NONE',  ( 14.37945523737839082, 2.499999999999745981, 7.667852709070308137 ) ) ;
#82261=CARTESIAN_POINT ( 'NONE',  ( -3.550000000000028244, 2.500000000000000000, -1.818653347947326138 ) ) ;
#82262=FACE_BOUND ( 'NONE', #111379, .T. ) ;
#82263=VERTEX_POINT ( 'NONE', #113242 ) ;
#82265=DIRECTION ( 'NONE',  ( -0.000000000000000000, -1.000000000000000000, -0.000000000000000000 ) ) ;
#82266=DIRECTION ( 'NONE',  ( -0.000000000000000000, 1.000000000000000000, -0.000000000000000000 ) ) ;
#82267=CIRCLE ( 'NONE', #78156, 0.1000000000000002554 ) ;
#82269=CARTESIAN_POINT ( 'NONE',  ( -5.850000000000018296, 12.50000000000000000, 1.537336459617582918 ) ) ;
#82272=VECTOR ( 'NONE', #30736, 1000.000000000000000 ) ;
#82273=AXIS2_PLACEMENT_3D ( 'NONE', #98353, #17865, #29623 ) ;
#82274=AXIS2_PLACEMENT_3D ( 'NONE', #99160, #19279, #59246 ) ;
#82275=CARTESIAN_POINT ( 'NONE',  ( -13.09999999999999254, 12.50000000000000000, -3.983716857408423628 ) ) ;
#82276=EDGE_LOOP ( 'NONE', ( #72259, #77095, #113463, #125754 ) ) ;
#82277=VERTEX_POINT ( 'NONE', #83789 ) ;
#82278=VERTEX_POINT ( 'NONE', #4549 ) ;
#82279=EDGE_LOOP ( 'NONE', ( #69164, #101477 ) ) ;
#82280=ORIENTED_EDGE ( 'NONE', *, *, #36423, .T. ) ;
#82281=DIRECTION ( 'NONE',  ( 0.000000000000000000, 1.000000000000000000, 0.000000000000000000 ) ) ;
#82282=DIRECTION ( 'NONE',  ( 0.000000000000000000, 0.000000000000000000, -1.000000000000000000 ) ) ;
#82283=EDGE_LOOP ( 'NONE', ( #116632, #80118 ) ) ;
#82284=FACE_BOUND ( 'NONE', #47050, .T. ) ;
#82285=AXIS2_PLACEMENT_3D ( 'NONE', #50163, #37753, #78979 ) ;
#82286=FACE_OUTER_BOUND ( 'NONE', #55760, .T. ) ;
#82287=AXIS2_PLACEMENT_3D ( 'NONE', #126080, #71334, #58652 ) ;
#82288=ADVANCED_FACE ( 'NONE', ( #124372 ), #30478, .T. ) ;
#82289=ADVANCED_FACE ( 'NONE', ( #5221 ), #97349, .T. ) ;
#82290=EDGE_LOOP ( 'NONE', ( #49996, #20969 ) ) ;
#82292=DIRECTION ( 'NONE',  ( 0.000000000000000000, 0.000000000000000000, 1.000000000000000000 ) ) ;
#82293=PLANE ( 'NONE',  #126925 ) ;
#82294=CONICAL_SURFACE ( 'NONE', #36342, 0.09999999999999999167, 0.003490658503988666988 ) ;
#82295=ORIENTED_EDGE ( 'NONE', *, *, #104336, .F. ) ;
#82296=CARTESIAN_POINT ( 'NONE',  ( -10.84999999999999964, 2.500000000000000000, 5.702370205355745014 ) ) ;
#82297=ORIENTED_EDGE ( 'NONE', *, *, #22526, .T. ) ;
#82298=AXIS2_PLACEMENT_3D ( 'NONE', #106236, #95767, #16537 ) ;
#82299=AXIS2_PLACEMENT_3D ( 'NONE', #21837, #82021, #110833 ) ;
#82300=AXIS2_PLACEMENT_3D ( 'NONE', #85532, #14827, #34522 ) ;
#82301=ORIENTED_EDGE ( 'NONE', *, *, #32334, .T. ) ;
#82302=ORIENTED_EDGE ( 'NONE', *, *, #34812, .F. ) ;
#82303=DIRECTION ( 'NONE',  ( -0.000000000000000000, -1.000000000000000000, -0.000000000000000000 ) ) ;
#82304=PLANE ( 'NONE',  #33073 ) ;
#82305=DIRECTION ( 'NONE',  ( -0.000000000000000000, 1.000000000000000000, -0.000000000000000000 ) ) ;
#82306=VECTOR ( 'NONE', #11440, 1000.000000000000000 ) ;
#82307=VERTEX_POINT ( 'NONE', #114528 ) ;
#82308=DIRECTION ( 'NONE',  ( -0.000000000000000000, -1.000000000000000000, -0.000000000000000000 ) ) ;
#82309=CIRCLE ( 'NONE', #15372, 0.06509327318403745899 ) ;
#82310=DIRECTION ( 'NONE',  ( 0.000000000000000000, 0.000000000000000000, 1.000000000000000000 ) ) ;
#82311=DIRECTION ( 'NONE',  ( 0.000000000000000000, 1.000000000000000000, 0.000000000000000000 ) ) ;
#82312=DIRECTION ( 'NONE',  ( -0.000000000000000000, 1.000000000000000000, -0.000000000000000000 ) ) ;
#82313=DIRECTION ( 'NONE',  ( -0.000000000000000000, -1.000000000000000000, -0.000000000000000000 ) ) ;
#82314=ORIENTED_EDGE ( 'NONE', *, *, #85629, .F. ) ;
#82315=FACE_OUTER_BOUND ( 'NONE', #27183, .T. ) ;
#82316=ORIENTED_EDGE ( 'NONE', *, *, #18960, .T. ) ;
#82317=DIRECTION ( 'NONE',  ( 0.000000000000000000, 0.000000000000000000, 1.000000000000000000 ) ) ;
#82318=EDGE_LOOP ( 'NONE', ( #51698, #80584 ) ) ;
#82319=ORIENTED_EDGE ( 'NONE', *, *, #104981, .F. ) ;
#82320=CARTESIAN_POINT ( 'NONE',  ( 4.149999999999941735, 2.500000000000000000, -2.757883832488654097 ) ) ;
#82321=DIRECTION ( 'NONE',  ( 0.000000000000000000, 0.000000000000000000, 1.000000000000000000 ) ) ;
#82322=AXIS2_PLACEMENT_3D ( 'NONE', #41145, #9079, #1193 ) ;
#82323=CARTESIAN_POINT ( 'NONE',  ( -12.29999999999999538, 2.500000000000000000, -0.2464101615137742063 ) ) ;
#82324=VECTOR ( 'NONE', #115099, 1000.000000000000000 ) ;
#82325=CARTESIAN_POINT ( 'NONE',  ( 12.09999999999990550, 2.500000000000000000, 4.230127018922196669 ) ) ;
#82326=CARTESIAN_POINT ( 'NONE',  ( 9.349999999999919709, 12.50000000000000000, 1.883746621131358934 ) ) ;
#82327=VERTEX_POINT ( 'NONE', #24876 ) ;
#82328=ORIENTED_EDGE ( 'NONE', *, *, #47169, .F. ) ;
#82329=ADVANCED_FACE ( 'NONE', ( #45170 ), #53053, .T. ) ;
#82330=DIRECTION ( 'NONE',  ( 0.000000000000000000, 1.000000000000000000, 0.000000000000000000 ) ) ;
#82331=VECTOR ( 'NONE', #74836, 1000.000000000000000 ) ;
#82332=AXIS2_PLACEMENT_3D ( 'NONE', #105860, #6984, #67859 ) ;
#82333=CIRCLE ( 'NONE', #101201, 0.06509327318403745899 ) ;
#82335=AXIS2_PLACEMENT_3D ( 'NONE', #12749, #110329, #31146 ) ;
#82336=CONICAL_SURFACE ( 'NONE', #96990, 0.09999999999999982514, 0.003490658503988666988 ) ;
#82337=CARTESIAN_POINT ( 'NONE',  ( 8.099999999999923261, 2.500000000000000000, 4.676537180435972552 ) ) ;
#82338=ORIENTED_EDGE ( 'NONE', *, *, #94451, .F. ) ;
#82339=EDGE_LOOP ( 'NONE', ( #104675, #9041, #62094, #39171 ) ) ;
#82340=ADVANCED_FACE ( 'NONE', ( #104706 ), #64146, .T. ) ;
#82341=CARTESIAN_POINT ( 'NONE',  ( 14.34999999999989662, 12.50000000000000000, 1.818653347947321475 ) ) ;
#82342=ORIENTED_EDGE ( 'NONE', *, *, #33121, .T. ) ;
#82343=DIRECTION ( 'NONE',  ( 0.000000000000000000, 0.000000000000000000, 1.000000000000000000 ) ) ;
#82344=ADVANCED_FACE ( 'NONE', ( #92982 ), #35347, .T. ) ;
#82345=DIRECTION ( 'NONE',  ( 0.000000000000000000, 1.000000000000000000, 0.000000000000000000 ) ) ;
#82346=AXIS2_PLACEMENT_3D ( 'NONE', #21532, #90248, #586 ) ;
#82348=CONICAL_SURFACE ( 'NONE', #38437, 0.1000000000000000472, 0.003490658503988666988 ) ;
#82349=CARTESIAN_POINT ( 'NONE',  ( -2.700000000000029932, 2.500000000000000000, -0.3464101615137782364 ) ) ;
#82350=ORIENTED_EDGE ( 'NONE', *, *, #76312, .F. ) ;
#82351=DIRECTION ( 'NONE',  ( 0.000000000000000000, -0.000000000000000000, 1.000000000000000000 ) ) ;
#82352=LINE ( 'NONE', #81056, #44541 ) ;
#82353=DIRECTION ( 'NONE',  ( 0.000000000000000000, 1.000000000000000000, 0.000000000000000000 ) ) ;
#82354=CARTESIAN_POINT ( 'NONE',  ( -10.60000000000000320, 2.500000000000000000, -4.676537180435973440 ) ) ;
#82355=VECTOR ( 'NONE', #43248, 1000.000000000000000 ) ;
#82356=EDGE_CURVE ( 'NONE', #69398, #91341, #113799, .T. ) ;
#82358=DIRECTION ( 'NONE',  ( 0.000000000000000000, 1.000000000000000000, 0.000000000000000000 ) ) ;
#82359=ORIENTED_EDGE ( 'NONE', *, *, #87414, .F. ) ;
#82360=DIRECTION ( 'NONE',  ( -0.000000000000000000, 1.000000000000000000, -0.000000000000000000 ) ) ;
#82361=PLANE ( 'NONE',  #102075 ) ;
#82362=ORIENTED_EDGE ( 'NONE', *, *, #73614, .T. ) ;
#82363=ORIENTED_EDGE ( 'NONE', *, *, #121501, .T. ) ;
#82364=EDGE_CURVE ( 'NONE', #53599, #11772, #16315, .T. ) ;
#82366=DIRECTION ( 'NONE',  ( 0.000000000000000000, 0.000000000000000000, -1.000000000000000000 ) ) ;
#82367=CARTESIAN_POINT ( 'NONE',  ( -2.950000000000029932, 2.500000000000000000, 2.165063509461097713 ) ) ;
#82368=CIRCLE ( 'NONE', #25919, 0.09999999999999982514 ) ;
#82369=DIRECTION ( 'NONE',  ( 0.000000000000000000, 1.000000000000000000, 0.000000000000000000 ) ) ;
#82370=DIRECTION ( 'NONE',  ( 0.000000000000000000, 1.000000000000000000, 0.000000000000000000 ) ) ;
#82371=DIRECTION ( 'NONE',  ( 0.000000000000000000, 1.000000000000000000, 0.000000000000000000 ) ) ;
#82372=DIRECTION ( 'NONE',  ( -0.000000000000000000, 1.000000000000000000, -0.000000000000000000 ) ) ;
#82373=PLANE ( 'NONE',  #91666 ) ;
#82374=B_SPLINE_CURVE_WITH_KNOTS ( 'NONE', 3,
 ( #129588, #11055, #39909, #58894, #121029, #30741, #31374, #40562, #101400, #80483, #121665, #32026 ),
 .UNSPECIFIED., .F., .F.,
 ( 4, 2, 2, 2, 2, 4 ),
 ( 3.476216610979977084E-18, 0.001300228439403502360, 0.002600456878807001250, 0.003900685318210500574, 0.004550799537912254139, 0.005200913757614008572 ),
 .UNSPECIFIED. ) ;
#82375=DIRECTION ( 'NONE',  ( -4.274815082592931898E-19, -0.9999939076577903929, -0.003490651415223739937 ) ) ;
#82376=AXIS2_PLACEMENT_3D ( 'NONE', #85167, #55705, #36075 ) ;
#82377=ORIENTED_EDGE ( 'NONE', *, *, #11407, .T. ) ;
#82378=VECTOR ( 'NONE', #66141, 1000.000000000000000 ) ;
#82379=EDGE_LOOP ( 'NONE', ( #18139, #66842 ) ) ;
#82380=EDGE_LOOP ( 'NONE', ( #122904, #77397, #63921, #66375 ) ) ;
#82381=EDGE_LOOP ( 'NONE', ( #93438, #19287, #58394, #80735 ) ) ;
#82382=AXIS2_PLACEMENT_3D ( 'NONE', #118315, #21400, #32541 ) ;
#82383=LINE ( 'NONE', #70611, #85899 ) ;
#82384=DIRECTION ( 'NONE',  ( -0.000000000000000000, 1.000000000000000000, -0.000000000000000000 ) ) ;
#82385=CIRCLE ( 'NONE', #65636, 0.06509327318403741736 ) ;
#82386=ORIENTED_EDGE ( 'NONE', *, *, #85625, .T. ) ;
#82387=DIRECTION ( 'NONE',  ( -0.000000000000000000, 1.000000000000000000, -0.000000000000000000 ) ) ;
#82388=CIRCLE ( 'NONE', #71924, 0.06509327318403745899 ) ;
#82389=EDGE_CURVE ( 'NONE', #49015, #48086, #17618, .T. ) ;
#82390=DIRECTION ( 'NONE',  ( 0.000000000000000000, 1.000000000000000000, 0.000000000000000000 ) ) ;
#82391=DIRECTION ( 'NONE',  ( 0.000000000000000000, 0.000000000000000000, -1.000000000000000000 ) ) ;
#82392=ORIENTED_EDGE ( 'NONE', *, *, #129062, .T. ) ;
#82393=ADVANCED_FACE ( 'NONE', ( #87645 ), #126301, .T. ) ;
#82394=CARTESIAN_POINT ( 'NONE',  ( 7.899999999999924860, 2.500000000000000000, -3.637306695894650055 ) ) ;
#82395=EDGE_CURVE ( 'NONE', #1004, #53300, #84641, .T. ) ;
#82396=CARTESIAN_POINT ( 'NONE',  ( 7.899999999999923084, 12.50000000000000000, -0.7579135962115917113 ) ) ;
#82397=VERTEX_POINT ( 'NONE', #18270 ) ;
#82398=AXIS2_PLACEMENT_3D ( 'NONE', #15904, #85295, #106856 ) ;
#82399=AXIS2_PLACEMENT_3D ( 'NONE', #91333, #29841, #10199 ) ;
#82400=EDGE_LOOP ( 'NONE', ( #70585, #97626 ) ) ;
#82401=EDGE_LOOP ( 'NONE', ( #19951, #33921 ) ) ;
#82402=EDGE_LOOP ( 'NONE', ( #128694, #34657, #43764, #60436 ) ) ;
#82403=DIRECTION ( 'NONE',  ( 0.000000000000000000, 0.000000000000000000, -1.000000000000000000 ) ) ;
#82404=EDGE_CURVE ( 'NONE', #79607, #120619, #101374, .T. ) ;
#82405=ADVANCED_FACE ( 'NONE', ( #96823 ), #1013, .T. ) ;
#82406=AXIS2_PLACEMENT_3D ( 'NONE', #118013, #59109, #116719 ) ;
#82407=ADVANCED_FACE ( 'NONE', ( #126948 ), #90899, .T. ) ;
#82408=ADVANCED_FACE ( 'NONE', ( #16944 ), #11479, .T. ) ;
#82409=DIRECTION ( 'NONE',  ( 0.000000000000000000, 0.000000000000000000, 1.000000000000000000 ) ) ;
#82410=DIRECTION ( 'NONE',  ( 0.000000000000000000, 0.000000000000000000, 1.000000000000000000 ) ) ;
#82411=CONICAL_SURFACE ( 'NONE', #122108, 0.1000000000000002554, 0.003490658503988666988 ) ;
#82412=DIRECTION ( 'NONE',  ( 0.000000000000000000, 1.000000000000000000, 0.000000000000000000 ) ) ;
#82413=ORIENTED_EDGE ( 'NONE', *, *, #124652, .T. ) ;
#82414=EDGE_CURVE ( 'NONE', #41903, #98295, #97162, .T. ) ;
#82416=VERTEX_POINT ( 'NONE', #75900 ) ;
#82417=FACE_OUTER_BOUND ( 'NONE', #122331, .T. ) ;
#82418=CARTESIAN_POINT ( 'NONE',  ( -8.350000000000013856, 2.500000000000000000, -2.165063509461101710 ) ) ;
#82419=DIRECTION ( 'NONE',  ( 0.000000000000000000, -0.9999939076577903929, 0.003490651415223739937 ) ) ;
#82420=DIRECTION ( 'NONE',  ( -0.000000000000000000, -1.000000000000000000, -0.000000000000000000 ) ) ;
#82421=EDGE_CURVE ( 'NONE', #58918, #71342, #15677, .T. ) ;
#82422=ORIENTED_EDGE ( 'NONE', *, *, #11145, .T. ) ;
#82423=ORIENTED_EDGE ( 'NONE', *, *, #26059, .T. ) ;
#82424=EDGE_LOOP ( 'NONE', ( #66244, #7537 ) ) ;
#82425=CARTESIAN_POINT ( 'NONE',  ( 6.649999999999930189, 12.50000000000000000, -2.922977105672691422 ) ) ;
#82426=DIRECTION ( 'NONE',  ( -0.000000000000000000, -1.000000000000000000, -0.000000000000000000 ) ) ;
#82427=DIRECTION ( 'NONE',  ( -0.000000000000000000, -1.000000000000000000, -0.000000000000000000 ) ) ;
#82428=FACE_BOUND ( 'NONE', #79526, .T. ) ;
#82429=PLANE ( 'NONE',  #38949 ) ;
#82430=CARTESIAN_POINT ( 'NONE',  ( 9.399999999999915090, 2.500000000000000000, -4.576537180435977348 ) ) ;
#82431=CARTESIAN_POINT ( 'NONE',  ( 11.84999999999990727, 2.500000000000000000, 6.741600689897071952 ) ) ;
#82432=CIRCLE ( 'NONE', #30200, 0.06509327318403745899 ) ;
#82433=AXIS2_PLACEMENT_3D ( 'NONE', #81558, #59359, #11521 ) ;
#82434=VECTOR ( 'NONE', #3496, 1000.000000000000000 ) ;
#82435=CONICAL_SURFACE ( 'NONE', #21794, 0.1000000000000002554, 0.003490658503988666988 ) ;
#82438=CARTESIAN_POINT ( 'NONE',  ( -7.500000000000001776, 2.500000000000000000, -9.000000000000000000 ) ) ;
#82439=ORIENTED_EDGE ( 'NONE', *, *, #97775, .F. ) ;
#82440=CIRCLE ( 'NONE', #82136, 0.06509327318403745899 ) ;
#82441=CARTESIAN_POINT ( 'NONE',  ( 4.599999999999938360, 12.50000000000000000, -0.6928203230275541413 ) ) ;
#82442=AXIS2_PLACEMENT_3D ( 'NONE', #118398, #28748, #68657 ) ;
#82443=AXIS2_PLACEMENT_3D ( 'NONE', #49933, #88533, #38834 ) ;
#82444=DIRECTION ( 'NONE',  ( -0.000000000000000000, -1.000000000000000000, -0.000000000000000000 ) ) ;
#82445=ORIENTED_EDGE ( 'NONE', *, *, #51808, .F. ) ;
#82446=ORIENTED_EDGE ( 'NONE', *, *, #82073, .T. ) ;
#82447=CIRCLE ( 'NONE', #3011, 0.1000000000000000472 ) ;
#82448=CARTESIAN_POINT ( 'NONE',  ( 1.449999999999952216, 2.500000000000000000, 1.818653347947321475 ) ) ;
#82449=DIRECTION ( 'NONE',  ( 0.000000000000000000, 0.000000000000000000, -1.000000000000000000 ) ) ;
#82450=FACE_BOUND ( 'NONE', #76842, .T. ) ;
#82451=CARTESIAN_POINT ( 'NONE',  ( -0.8500000000000386136, 2.500000000000000000, 5.702370205355745014 ) ) ;
#82452=EDGE_CURVE ( 'NONE', #109690, #45787, #55396, .T. ) ;
#82453=VERTEX_POINT ( 'NONE', #77827 ) ;
#82454=CARTESIAN_POINT ( 'NONE',  ( -12.04999999999999716, 12.50000000000000000, -6.560283801567336148 ) ) ;
#82455=CARTESIAN_POINT ( 'NONE',  ( -4.200000000000029488, 2.500000000000000000, -4.330127018922201643 ) ) ;
#82456=VECTOR ( 'NONE', #97532, 1000.000000000000000 ) ;
#82457=ORIENTED_EDGE ( 'NONE', *, *, #126681, .T. ) ;
#82458=CARTESIAN_POINT ( 'NONE',  ( 0.8499999999999536815, 12.50000000000000000, 6.495190528383297135 ) ) ;
#82459=CARTESIAN_POINT ( 'NONE',  ( 11.44999999999990692, 2.500000000000000000, 1.818653347947321475 ) ) ;
#82460=EDGE_CURVE ( 'NONE', #75963, #92171, #66717, .T. ) ;
#82461=ORIENTED_EDGE ( 'NONE', *, *, #84315, .F. ) ;
#82462=FACE_OUTER_BOUND ( 'NONE', #70130, .T. ) ;
#82463=DIRECTION ( 'NONE',  ( -0.000000000000000000, 1.000000000000000000, -0.000000000000000000 ) ) ;
#82464=CIRCLE ( 'NONE', #71994, 0.1000000000000000056 ) ;
#82465=ORIENTED_EDGE ( 'NONE', *, *, #16327, .F. ) ;
#82466=CARTESIAN_POINT ( 'NONE',  ( -7.050000000000013145, 2.500000000000000000, 6.495190528383297135 ) ) ;
#82467=DIRECTION ( 'NONE',  ( -0.000000000000000000, 1.000000000000000000, -0.000000000000000000 ) ) ;
#82468=CARTESIAN_POINT ( 'NONE',  ( -7.100000000000017408, 12.50000000000000000, -0.6277270498435167934 ) ) ;
#82469=VERTEX_POINT ( 'NONE', #47109 ) ;
#82470=EDGE_LOOP ( 'NONE', ( #4113, #122579, #73096, #128873 ) ) ;
#82471=DIRECTION ( 'NONE',  ( 0.000000000000000000, -0.9999939076577903929, 0.003490651415223739937 ) ) ;
#82472=EDGE_LOOP ( 'NONE', ( #83224, #19523 ) ) ;
#82473=DIRECTION ( 'NONE',  ( 0.000000000000000000, 1.000000000000000000, 0.000000000000000000 ) ) ;
#82474=DIRECTION ( 'NONE',  ( -0.000000000000000000, 1.000000000000000000, -0.000000000000000000 ) ) ;
#82475=AXIS2_PLACEMENT_3D ( 'NONE', #89948, #29122, #82063 ) ;
#82476=CARTESIAN_POINT ( 'NONE',  ( 3.349999999999944578, 2.500000000000000000, -1.572243186433550211 ) ) ;
#82477=ORIENTED_EDGE ( 'NONE', *, *, #113582, .F. ) ;
#82478=CARTESIAN_POINT ( 'NONE',  ( -13.74999999999998757, 2.500000000000000000, 1.372243186433549367 ) ) ;
#82479=FACE_OUTER_BOUND ( 'NONE', #42402, .T. ) ;
#82480=CARTESIAN_POINT ( 'NONE',  ( 11.64999999999990798, 2.500000000000000000, -2.857883832488653741 ) ) ;
#82481=CARTESIAN_POINT ( 'NONE',  ( -12.69999999999999041, 2.500000000000000000, 3.883716857408421319 ) ) ;
#82482=CARTESIAN_POINT ( 'NONE',  ( 6.699999999999930012, 2.500000000000000000, -4.230127018922201998 ) ) ;
#82483=CARTESIAN_POINT ( 'NONE',  ( 11.24999999999990763, 12.50000000000000000, -7.122917578226816815 ) ) ;
#82484=VERTEX_POINT ( 'NONE', #67336 ) ;
#82485=EDGE_CURVE ( 'NONE', #112225, #69443, #103426, .T. ) ;
#82486=EDGE_LOOP ( 'NONE', ( #35717, #67899 ) ) ;
#82487=DIRECTION ( 'NONE',  ( 0.000000000000000000, 0.000000000000000000, 1.000000000000000000 ) ) ;
#82488=EDGE_LOOP ( 'NONE', ( #25140, #14666, #29667, #51078 ) ) ;
#82489=AXIS2_PLACEMENT_3D ( 'NONE', #116873, #27217, #65188 ) ;
#82490=DIRECTION ( 'NONE',  ( 0.000000000000000000, 0.000000000000000000, 1.000000000000000000 ) ) ;
#82491=ORIENTED_EDGE ( 'NONE', *, *, #90344, .T. ) ;
#82492=ORIENTED_EDGE ( 'NONE', *, *, #60539, .F. ) ;
#82493=ORIENTED_EDGE ( 'NONE', *, *, #10106, .T. ) ;
#82494=AXIS2_PLACEMENT_3D ( 'NONE', #51868, #31578, #102254 ) ;
#82495=CARTESIAN_POINT ( 'NONE',  ( -11.25000000000000000, 12.50000000000000000, 7.253104124594885960 ) ) ;
#82496=VECTOR ( 'NONE', #88697, 1000.000000000000000 ) ;
#82497=DIRECTION ( 'NONE',  ( 0.000000000000000000, 1.000000000000000000, 0.000000000000000000 ) ) ;
#82498=ADVANCED_FACE ( 'NONE', ( #28098 ), #21967, .T. ) ;
#82499=CARTESIAN_POINT ( 'NONE',  ( 12.49999999999993960, 12.50000000000000000, 4.395220292106234439 ) ) ;
#82500=FACE_OUTER_BOUND ( 'NONE', #31771, .T. ) ;
#82502=DIRECTION ( 'NONE',  ( 0.000000000000000000, 0.000000000000000000, -1.000000000000000000 ) ) ;
#82503=CARTESIAN_POINT ( 'NONE',  ( -1.250000000000037970, 12.50000000000000000, 2.857883832488649301 ) ) ;
#82504=DIRECTION ( 'NONE',  ( 0.000000000000000000, 0.000000000000000000, -1.000000000000000000 ) ) ;
#82505=EDGE_CURVE ( 'NONE', #129541, #43692, #51201, .T. ) ;
#82506=EDGE_CURVE ( 'NONE', #89650, #57903, #118082, .T. ) ;
#82507=DIRECTION ( 'NONE',  ( 0.000000000000000000, -0.000000000000000000, 1.000000000000000000 ) ) ;
#82508=ORIENTED_EDGE ( 'NONE', *, *, #115525, .F. ) ;
#82509=EDGE_CURVE ( 'NONE', #16531, #121848, #24005, .T. ) ;
#82510=CIRCLE ( 'NONE', #115941, 0.06509327318403745899 ) ;
#82511=FACE_OUTER_BOUND ( 'NONE', #96834, .T. ) ;
#82512=CIRCLE ( 'NONE', #59548, 0.09999999999999982514 ) ;
#82513=AXIS2_PLACEMENT_3D ( 'NONE', #114329, #56044, #64581 ) ;
#82514=ORIENTED_EDGE ( 'NONE', *, *, #124578, .F. ) ;
#82515=EDGE_LOOP ( 'NONE', ( #107581, #8749 ) ) ;
#82516=ADVANCED_FACE ( 'NONE', ( #36650 ), #76553, .T. ) ;
#82517=DIRECTION ( 'NONE',  ( 0.000000000000000000, 0.000000000000000000, -1.000000000000000000 ) ) ;
#82518=CARTESIAN_POINT ( 'NONE',  ( 5.399999999999932854, 2.500000000000000000, 5.122947341949749323 ) ) ;
#82519=DIRECTION ( 'NONE',  ( -0.000000000000000000, 1.000000000000000000, -0.000000000000000000 ) ) ;
#82520=AXIS2_PLACEMENT_3D ( 'NONE', #49024, #88932, #128884 ) ;
#82521=CARTESIAN_POINT ( 'NONE',  ( 0.6499999999999566125, 2.500000000000000000, -6.841600689897077814 ) ) ;
#82522=CIRCLE ( 'NONE', #11679, 0.09999999999999982514 ) ;
#82523=DIRECTION ( 'NONE',  ( 0.000000000000000000, 0.000000000000000000, -1.000000000000000000 ) ) ;
#82524=CARTESIAN_POINT ( 'NONE',  ( -12.69999999999999218, 12.50000000000000000, -0.3464101615137741286 ) ) ;
#82525=CARTESIAN_POINT ( 'NONE',  ( -17.50000000000000000, -1.500000000000000000, 1.734723475976807094E-15 ) ) ;
#82526=ORIENTED_EDGE ( 'NONE', *, *, #111009, .F. ) ;
#82527=CIRCLE ( 'NONE', #26081, 0.06509327318403745899 ) ;
#82528=CONICAL_SURFACE ( 'NONE', #88775, 0.1000000000000000472, 0.003490658503988666988 ) ;
#82529=ORIENTED_EDGE ( 'NONE', *, *, #75159, .T. ) ;
#82530=AXIS2_PLACEMENT_3D ( 'NONE', #6415, #44445, #43825 ) ;
#82531=VERTEX_POINT ( 'NONE', #79148 ) ;
#82532=VERTEX_POINT ( 'NONE', #60783 ) ;
#82533=CIRCLE ( 'NONE', #26095, 0.06509327318403745899 ) ;
#82534=VERTEX_POINT ( 'NONE', #553 ) ;
#82535=LINE ( 'NONE', #40028, #85805 ) ;
#82536=CARTESIAN_POINT ( 'NONE',  ( -10.60000000000000142, 12.50000000000000000, -0.3464101615137782364 ) ) ;
#82538=CARTESIAN_POINT ( 'NONE',  ( -5.800000000000018474, 12.50000000000000000, -0.06509327318403970719 ) ) ;
#82539=DIRECTION ( 'NONE',  ( 0.000000000000000000, 0.000000000000000000, 1.000000000000000000 ) ) ;
#82541=CARTESIAN_POINT ( 'NONE',  ( -0.6500000000000398792, 2.500000000000000000, -2.511473670974877948 ) ) ;
#82542=DIRECTION ( 'NONE',  ( -0.000000000000000000, 1.000000000000000000, -0.000000000000000000 ) ) ;
#82543=DIRECTION ( 'NONE',  ( 0.000000000000000000, 1.000000000000000000, 0.000000000000000000 ) ) ;
#82544=AXIS2_PLACEMENT_3D ( 'NONE', #15194, #66964, #35604 ) ;
#82546=ORIENTED_EDGE ( 'NONE', *, *, #101552, .T. ) ;
#82547=ORIENTED_EDGE ( 'NONE', *, *, #36538, .T. ) ;
#82548=VERTEX_POINT ( 'NONE', #18904 ) ;
#82549=EDGE_CURVE ( 'NONE', #71852, #115126, #61665, .T. ) ;
#82550=DIRECTION ( 'NONE',  ( 0.000000000000000000, 1.000000000000000000, 0.000000000000000000 ) ) ;
#82551=EDGE_CURVE ( 'NONE', #27445, #22099, #100065, .T. ) ;
#82552=EDGE_CURVE ( 'NONE', #43625, #94349, #28208, .T. ) ;
#82553=EDGE_LOOP ( 'NONE', ( #109423, #18258 ) ) ;
#82554=AXIS2_PLACEMENT_3D ( 'NONE', #93889, #34341, #15297 ) ;
#82555=EDGE_CURVE ( 'NONE', #8533, #79987, #9325, .T. ) ;
#82556=DIRECTION ( 'NONE',  ( -0.000000000000000000, 1.000000000000000000, -0.000000000000000000 ) ) ;
#82557=CARTESIAN_POINT ( 'NONE',  ( 3.349999999999945466, 2.500000000000000000, -2.065063509461102065 ) ) ;
#82558=CIRCLE ( 'NONE', #44994, 0.06509327318403745899 ) ;
#82559=EDGE_CURVE ( 'NONE', #94388, #129360, #105573, .T. ) ;
#82560=EDGE_LOOP ( 'NONE', ( #71365, #73243 ) ) ;
#82561=DIRECTION ( 'NONE',  ( 0.000000000000000000, 0.000000000000000000, 1.000000000000000000 ) ) ;
#82562=DIRECTION ( 'NONE',  ( 0.000000000000000000, 0.000000000000000000, -1.000000000000000000 ) ) ;
#82564=DIRECTION ( 'NONE',  ( 0.000000000000000000, 0.000000000000000000, 1.000000000000000000 ) ) ;
#82565=EDGE_CURVE ( 'NONE', #51534, #110814, #49063, .T. ) ;
#82566=AXIS2_PLACEMENT_3D ( 'NONE', #86569, #27023, #58426 ) ;
#82567=EDGE_CURVE ( 'NONE', #24704, #38510, #78395, .T. ) ;
#82568=CARTESIAN_POINT ( 'NONE',  ( -11.69999999999999929, 12.50000000000000000, 0.06509327318403916596 ) ) ;
#82569=CIRCLE ( 'NONE', #22026, 0.1000000000000002554 ) ;
#82570=EDGE_LOOP ( 'NONE', ( #90977, #13003, #83943, #118338 ) ) ;
#82571=ORIENTED_EDGE ( 'NONE', *, *, #28903, .T. ) ;
#82572=LINE ( 'NONE', #62916, #91932 ) ;
#82573=DIRECTION ( 'NONE',  ( 0.000000000000000000, 0.000000000000000000, 1.000000000000000000 ) ) ;
#82574=ADVANCED_FACE ( 'NONE', ( #90218 ), #111838, .T. ) ;
#82575=CARTESIAN_POINT ( 'NONE',  ( 1.849999999999950573, 12.50000000000000000, 2.446380397790835826 ) ) ;
#82576=DIRECTION ( 'NONE',  ( 0.000000000000000000, 1.000000000000000000, 0.000000000000000000 ) ) ;
#82577=VERTEX_POINT ( 'NONE', #111143 ) ;
#82578=AXIS2_PLACEMENT_3D ( 'NONE', #12381, #71971, #41229 ) ;
#82579=CIRCLE ( 'NONE', #11459, 0.1000000000000000472 ) ;
#82580=ORIENTED_EDGE ( 'NONE', *, *, #49089, .T. ) ;
#82581=CARTESIAN_POINT ( 'NONE',  ( -3.950000000000026379, 2.500000000000000000, -1.918653347947326004 ) ) ;
#82582=DIRECTION ( 'NONE',  ( 0.000000000000000000, 0.000000000000000000, 1.000000000000000000 ) ) ;
#82583=DIRECTION ( 'NONE',  ( 0.000000000000000000, 1.000000000000000000, 0.000000000000000000 ) ) ;
#82584=LINE ( 'NONE', #13160, #92735 ) ;
#82585=ORIENTED_EDGE ( 'NONE', *, *, #109271, .F. ) ;
#82586=CARTESIAN_POINT ( 'NONE',  ( 9.549999999999918998, 12.50000000000000000, -6.560283801567339701 ) ) ;
#82587=CARTESIAN_POINT ( 'NONE',  ( 11.44999999999990692, 12.50000000000000000, 1.818653347947321475 ) ) ;
#82588=ORIENTED_EDGE ( 'NONE', *, *, #93067, .F. ) ;
#82589=LINE ( 'NONE', #70817, #9308 ) ;
#82591=ORIENTED_EDGE ( 'NONE', *, *, #22829, .T. ) ;
#82592=CARTESIAN_POINT ( 'NONE',  ( 6.649999999999930189, 12.50000000000000000, -2.792790559304616504 ) ) ;
#82593=CIRCLE ( 'NONE', #36636, 0.06509327318403745899 ) ;
#82594=EDGE_LOOP ( 'NONE', ( #1147, #58501 ) ) ;
#82595=DIRECTION ( 'NONE',  ( 0.000000000000000000, 0.000000000000000000, -1.000000000000000000 ) ) ;
#82596=CARTESIAN_POINT ( 'NONE',  ( -6.450000000000019718, 2.500000000000000000, -1.718653347947326049 ) ) ;
#82597=CIRCLE ( 'NONE', #55400, 0.1000000000000002554 ) ;
#82598=ORIENTED_EDGE ( 'NONE', *, *, #342, .T. ) ;
#82599=ORIENTED_EDGE ( 'NONE', *, *, #77747, .F. ) ;
#82601=FACE_OUTER_BOUND ( 'NONE', #45373, .T. ) ;
#82604=AXIS2_PLACEMENT_3D ( 'NONE', #25326, #5685, #16780 ) ;
#82605=EDGE_CURVE ( 'NONE', #117649, #115225, #95110, .T. ) ;
#82606=CIRCLE ( 'NONE', #92980, 0.1000000000000002554 ) ;
#82607=DIRECTION ( 'NONE',  ( -4.274815082592931898E-19, -0.9999939076577903929, -0.003490651415223739937 ) ) ;
#82608=LINE ( 'NONE', #41401, #17964 ) ;
#82609=DIRECTION ( 'NONE',  ( 0.000000000000000000, 1.000000000000000000, 0.000000000000000000 ) ) ;
#82610=AXIS2_PLACEMENT_3D ( 'NONE', #33293, #73198, #113113 ) ;
#82611=LINE ( 'NONE', #30299, #68230 ) ;
#82612=PLANE ( 'NONE',  #14899 ) ;
#82613=CIRCLE ( 'NONE', #74295, 0.06509327318403745899 ) ;
#82614=AXIS2_PLACEMENT_3D ( 'NONE', #86942, #110922, #77755 ) ;
#82615=EDGE_LOOP ( 'NONE', ( #13055, #95972 ) ) ;
#82616=ORIENTED_EDGE ( 'NONE', *, *, #2690, .T. ) ;
#82617=CARTESIAN_POINT ( 'NONE',  ( -2.050000000000033129, 2.500000000000000000, 6.495190528383297135 ) ) ;
#82618=VERTEX_POINT ( 'NONE', #21497 ) ;
#82619=DIRECTION ( 'NONE',  ( -0.000000000000000000, -1.000000000000000000, -0.000000000000000000 ) ) ;
#82620=PLANE ( 'NONE',  #7387 ) ;
#82621=CONICAL_SURFACE ( 'NONE', #101396, 0.1000000000000000472, 0.003490658503988666988 ) ;
#82622=DIRECTION ( 'NONE',  ( -0.000000000000000000, 1.000000000000000000, -0.000000000000000000 ) ) ;
#82623=ORIENTED_EDGE ( 'NONE', *, *, #27842, .F. ) ;
#82624=ORIENTED_EDGE ( 'NONE', *, *, #16590, .F. ) ;
#82625=FACE_BOUND ( 'NONE', #49175, .T. ) ;
#82626=EDGE_LOOP ( 'NONE', ( #65733, #40318, #59220, #56847 ) ) ;
#82627=DIRECTION ( 'NONE',  ( 0.000000000000000000, 1.000000000000000000, 0.000000000000000000 ) ) ;
#82628=CARTESIAN_POINT ( 'NONE',  ( 7.499999999999961808, 2.500000000000000000, 4.230127018922196669 ) ) ;
#82629=DIRECTION ( 'NONE',  ( 0.000000000000000000, 0.000000000000000000, 1.000000000000000000 ) ) ;
#82630=CARTESIAN_POINT ( 'NONE',  ( 12.49999999999993960, 2.500000000000000000, 4.330127018922196314 ) ) ;
#82631=DIRECTION ( 'NONE',  ( 0.000000000000000000, 1.000000000000000000, 0.000000000000000000 ) ) ;
#82632=PLANE ( 'NONE',  #6845 ) ;
#82633=DIRECTION ( 'NONE',  ( -0.000000000000000000, 1.000000000000000000, -0.000000000000000000 ) ) ;
#82635=DIRECTION ( 'NONE',  ( 0.000000000000000000, 0.000000000000000000, 1.000000000000000000 ) ) ;
#82636=FACE_OUTER_BOUND ( 'NONE', #101002, .T. ) ;
#82637=CIRCLE ( 'NONE', #36581, 0.06509327318403745899 ) ;
#82638=DIRECTION ( 'NONE',  ( 0.000000000000000000, 0.000000000000000000, 1.000000000000000000 ) ) ;
#82639=ORIENTED_EDGE ( 'NONE', *, *, #7684, .T. ) ;
#82640=ORIENTED_EDGE ( 'NONE', *, *, #8362, .T. ) ;
#82641=EDGE_LOOP ( 'NONE', ( #1879, #120035 ) ) ;
#82642=CARTESIAN_POINT ( 'NONE',  ( -1.250000000000037970, 2.500000000000000000, 7.088010851410848190 ) ) ;
#82643=ORIENTED_EDGE ( 'NONE', *, *, #110678, .F. ) ;
#82644=DIRECTION ( 'NONE',  ( -0.000000000000000000, 1.000000000000000000, -0.000000000000000000 ) ) ;
#82645=EDGE_LOOP ( 'NONE', ( #15064, #51426 ) ) ;
#82647=CONICAL_SURFACE ( 'NONE', #111880, 0.1000000000000000472, 0.003490658503988666988 ) ;
#82648=ORIENTED_EDGE ( 'NONE', *, *, #108769, .T. ) ;
#82649=FACE_OUTER_BOUND ( 'NONE', #96330, .T. ) ;
#82650=CONICAL_SURFACE ( 'NONE', #124506, 0.1000000000000002554, 0.003490658503988666988 ) ;
#82651=VECTOR ( 'NONE', #69711, 1000.000000000000000 ) ;
#82652=ADVANCED_FACE ( 'NONE', ( #100687 ), #101358, .T. ) ;
#82653=DIRECTION ( 'NONE',  ( 0.000000000000000000, 1.000000000000000000, 0.000000000000000000 ) ) ;
#82654=DIRECTION ( 'NONE',  ( -0.000000000000000000, 1.000000000000000000, -0.000000000000000000 ) ) ;
#82655=DIRECTION ( 'NONE',  ( 0.000000000000000000, 1.000000000000000000, 0.000000000000000000 ) ) ;
#82656=DIRECTION ( 'NONE',  ( 0.000000000000000000, 0.000000000000000000, -1.000000000000000000 ) ) ;
#82657=ADVANCED_FACE ( 'NONE', ( #50977 ), #57454, .T. ) ;
#82658=ORIENTED_EDGE ( 'NONE', *, *, #49435, .F. ) ;
#82660=CARTESIAN_POINT ( 'NONE',  ( -10.60000000000000142, 12.50000000000000000, 4.048810130592458201 ) ) ;
#82661=ORIENTED_EDGE ( 'NONE', *, *, #98924, .F. ) ;
#82662=CIRCLE ( 'NONE', #93125, 0.1000000000000002554 ) ;
#82663=VERTEX_POINT ( 'NONE', #109216 ) ;
#82664=ORIENTED_EDGE ( 'NONE', *, *, #119469, .T. ) ;
#82665=VECTOR ( 'NONE', #25949, 1000.000000000000000 ) ;
#82666=ADVANCED_FACE ( 'NONE', ( #30695 ), #13522, .T. ) ;
#82668=ADVANCED_FACE ( 'NONE', ( #120990 ), #126409, .T. ) ;
#82669=EDGE_CURVE ( 'NONE', #110342, #37153, #49691, .T. ) ;
#82670=VERTEX_POINT ( 'NONE', #79774 ) ;
#82671=ORIENTED_EDGE ( 'NONE', *, *, #75973, .T. ) ;
#82672=ADVANCED_FACE ( 'NONE', ( #30043 ), #61766, .T. ) ;
#82673=EDGE_CURVE ( 'NONE', #98422, #29970, #30278, .T. ) ;
#82674=ORIENTED_EDGE ( 'NONE', *, *, #57810, .T. ) ;
#82676=DIRECTION ( 'NONE',  ( 0.000000000000000000, 0.000000000000000000, -1.000000000000000000 ) ) ;
#82677=AXIS2_PLACEMENT_3D ( 'NONE', #40253, #80171, #58607 ) ;
#82678=DIRECTION ( 'NONE',  ( 0.000000000000000000, -0.000000000000000000, 1.000000000000000000 ) ) ;
#82679=VECTOR ( 'NONE', #53166, 1000.000000000000000 ) ;
#82680=CARTESIAN_POINT ( 'NONE',  ( -6.250000000000021316, 2.500000000000000000, -1.572243186433550211 ) ) ;
#82681=CARTESIAN_POINT ( 'NONE',  ( -14.59999999999998366, 2.500000000000000000, -0.6928203230275520319 ) ) ;
#82682=CARTESIAN_POINT ( 'NONE',  ( -13.14999999999999147, 2.500000000000000000, -1.718653347947323828 ) ) ;
#82683=ADVANCED_FACE ( 'NONE', ( #3157 ), #9520, .T. ) ;
#82684=DIRECTION ( 'NONE',  ( 0.000000000000000000, 0.000000000000000000, -1.000000000000000000 ) ) ;
#82685=ORIENTED_EDGE ( 'NONE', *, *, #94049, .F. ) ;
#82686=DIRECTION ( 'NONE',  ( -0.000000000000000000, -1.000000000000000000, -0.000000000000000000 ) ) ;
#82687=ORIENTED_EDGE ( 'NONE', *, *, #33029, .T. ) ;
#82688=DIRECTION ( 'NONE',  ( 0.000000000000000000, 0.000000000000000000, 1.000000000000000000 ) ) ;
#82689=AXIS2_PLACEMENT_3D ( 'NONE', #31297, #70548, #60114 ) ;
#82690=VERTEX_POINT ( 'NONE', #4399 ) ;
#82691=FACE_OUTER_BOUND ( 'NONE', #8679, .T. ) ;
#82692=CIRCLE ( 'NONE', #120333, 0.09999999999999999167 ) ;
#82693=EDGE_LOOP ( 'NONE', ( #77427, #124832, #32426, #23047 ) ) ;
#82694=CARTESIAN_POINT ( 'NONE',  ( -1.900000000000034994, 2.500000000000000000, -0.2464101615137783419 ) ) ;
#82695=AXIS2_PLACEMENT_3D ( 'NONE', #84047, #24497, #113513 ) ;
#82696=AXIS2_PLACEMENT_3D ( 'NONE', #38930, #69642, #78844 ) ;
#82697=CARTESIAN_POINT ( 'NONE',  ( -12.69999999999999218, 2.500000000000000000, -4.676537180435975216 ) ) ;
#82698=ORIENTED_EDGE ( 'NONE', *, *, #5193, .F. ) ;
#82699=EDGE_LOOP ( 'NONE', ( #48563, #2151 ) ) ;
#82701=DIRECTION ( 'NONE',  ( -0.000000000000000000, 1.000000000000000000, -0.000000000000000000 ) ) ;
#82702=CARTESIAN_POINT ( 'NONE',  ( 0.8499999999999545697, 2.500000000000000000, -1.472243186433550122 ) ) ;
#82703=DIRECTION ( 'NONE',  ( 0.000000000000000000, 0.000000000000000000, 1.000000000000000000 ) ) ;
#82704=CARTESIAN_POINT ( 'NONE',  ( -11.64999999999999858, 12.50000000000000000, -1.472243186433546125 ) ) ;
#82705=AXIS2_PLACEMENT_3D ( 'NONE', #37441, #46595, #36144 ) ;
#82706=CARTESIAN_POINT ( 'NONE',  ( 7.699999999999923794, 2.500000000000000000, -4.083716857408426826 ) ) ;
#82707=ORIENTED_EDGE ( 'NONE', *, *, #84750, .T. ) ;
#82708=CARTESIAN_POINT ( 'NONE',  ( 2.500000000000002220, -2.500000000000000000, 9.261799387799150907 ) ) ;
#82709=VECTOR ( 'NONE', #54666, 1000.000000000000000 ) ;
#82710=EDGE_CURVE ( 'NONE', #3855, #3469, #43102, .T. ) ;
#82711=EDGE_CURVE ( 'NONE', #4247, #40133, #15757, .T. ) ;
#82712=ORIENTED_EDGE ( 'NONE', *, *, #39200, .F. ) ;
#82713=AXIS2_PLACEMENT_3D ( 'NONE', #120037, #91217, #70293 ) ;
#82714=DIRECTION ( 'NONE',  ( 0.000000000000000000, 0.000000000000000000, 1.000000000000000000 ) ) ;
#82715=CARTESIAN_POINT ( 'NONE',  ( 6.449999999999931788, 2.500000000000000000, -2.511473670974877948 ) ) ;
#82716=AXIS2_PLACEMENT_3D ( 'NONE', #95806, #76176, #125897 ) ;
#82717=ADVANCED_FACE ( 'NONE', ( #43743 ), #65850, .T. ) ;
#82718=AXIS2_PLACEMENT_3D ( 'NONE', #98397, #57858, #17909 ) ;
#82720=CARTESIAN_POINT ( 'NONE',  ( 0.3999999999999628852, 12.50000000000000000, -0.6928203230275520319 ) ) ;
#82721=DIRECTION ( 'NONE',  ( 0.000000000000000000, 0.000000000000000000, 1.000000000000000000 ) ) ;
#82722=ADVANCED_FACE ( 'NONE', ( #112469 ), #40846, .T. ) ;
#82723=CARTESIAN_POINT ( 'NONE',  ( 1.849999999999950129, 2.500000000000000000, -6.941600689897078347 ) ) ;
#82724=FACE_OUTER_BOUND ( 'NONE', #23809, .T. ) ;
#82725=VERTEX_POINT ( 'NONE', #102624 ) ;
#82726=EDGE_CURVE ( 'NONE', #20272, #72203, #28301, .T. ) ;
#82727=EDGE_CURVE ( 'NONE', #84568, #37944, #5293, .T. ) ;
#82728=DIRECTION ( 'NONE',  ( 0.000000000000000000, 0.000000000000000000, 1.000000000000000000 ) ) ;
#82729=EDGE_CURVE ( 'NONE', #74213, #48575, #95202, .T. ) ;
#82730=DIRECTION ( 'NONE',  ( 0.000000000000000000, 0.000000000000000000, 1.000000000000000000 ) ) ;
#82731=PLANE ( 'NONE',  #28720 ) ;
#82732=ORIENTED_EDGE ( 'NONE', *, *, #99502, .T. ) ;
#82733=AXIS2_PLACEMENT_3D ( 'NONE', #25598, #16407, #56990 ) ;
#82734=EDGE_CURVE ( 'NONE', #6628, #103260, #51307, .T. ) ;
#82735=CARTESIAN_POINT ( 'NONE',  ( -11.89999999999999680, 2.500000000000000000, 0.3464101615137776813 ) ) ;
#82736=VERTEX_POINT ( 'NONE', #33275 ) ;
#82737=ORIENTED_EDGE ( 'NONE', *, *, #116901, .F. ) ;
#82738=LINE ( 'NONE', #113462, #28034 ) ;
#82739=AXIS2_PLACEMENT_3D ( 'NONE', #10480, #39961, #32734 ) ;
#82740=ORIENTED_EDGE ( 'NONE', *, *, #23212, .T. ) ;
#82741=CARTESIAN_POINT ( 'NONE',  ( -3.550000000000028688, 2.500000000000000000, 6.741600689897071952 ) ) ;
#82742=DIRECTION ( 'NONE',  ( 0.000000000000000000, 1.000000000000000000, 0.000000000000000000 ) ) ;
#82743=LINE ( 'NONE', #124586, #119598 ) ;
#82744=AXIS2_PLACEMENT_3D ( 'NONE', #36266, #26440, #106280 ) ;
#82745=CIRCLE ( 'NONE', #122448, 0.1000000000000000472 ) ;
#82746=ORIENTED_EDGE ( 'NONE', *, *, #61118, .F. ) ;
#82747=DIRECTION ( 'NONE',  ( 0.000000000000000000, 0.000000000000000000, 1.000000000000000000 ) ) ;
#82748=CIRCLE ( 'NONE', #55545, 1.000000000000000888 ) ;
#82749=DIRECTION ( 'NONE',  ( -4.274815082592931898E-19, -0.9999939076577903929, -0.003490651415223739937 ) ) ;
#82750=EDGE_CURVE ( 'NONE', #66161, #92620, #7350, .T. ) ;
#82751=ORIENTED_EDGE ( 'NONE', *, *, #52568, .T. ) ;
#82752=AXIS2_PLACEMENT_3D ( 'NONE', #111874, #83065, #52957 ) ;
#82753=ORIENTED_EDGE ( 'NONE', *, *, #69128, .F. ) ;
#82754=AXIS2_PLACEMENT_3D ( 'NONE', #8556, #48504, #11139 ) ;
#82755=AXIS2_PLACEMENT_3D ( 'NONE', #18041, #107724, #87427 ) ;
#82756=VERTEX_POINT ( 'NONE', #13595 ) ;
#82757=FACE_OUTER_BOUND ( 'NONE', #119002, .T. ) ;
#82758=CARTESIAN_POINT ( 'NONE',  ( -7.900000000000014566, 2.500000000000000000, -4.230127018922201998 ) ) ;
#82759=DIRECTION ( 'NONE',  ( -4.274815082592931898E-19, -0.9999939076577903929, -0.003490651415223739937 ) ) ;
#82760=FACE_BOUND ( 'NONE', #15928, .T. ) ;
#82761=VERTEX_POINT ( 'NONE', #52896 ) ;
#82762=CARTESIAN_POINT ( 'NONE',  ( 5.799999999999931433, 12.50000000000000000, 4.330127018922196314 ) ) ;
#82763=DIRECTION ( 'NONE',  ( 0.000000000000000000, 0.000000000000000000, -1.000000000000000000 ) ) ;
#82764=ORIENTED_EDGE ( 'NONE', *, *, #14223, .F. ) ;
#82765=CARTESIAN_POINT ( 'NONE',  ( -11.89999999999999503, 12.50000000000000000, 4.741630453620009789 ) ) ;
#82766=CIRCLE ( 'NONE', #97327, 0.09999999999999982514 ) ;
#82767=FACE_OUTER_BOUND ( 'NONE', #105497, .T. ) ;
#82768=CONICAL_SURFACE ( 'NONE', #78564, 0.1000000000000000472, 0.003490658503988666988 ) ;
#82769=EDGE_CURVE ( 'NONE', #11681, #55449, #123547, .T. ) ;
#82770=FACE_OUTER_BOUND ( 'NONE', #76271, .T. ) ;
#82771=DIRECTION ( 'NONE',  ( 0.000000000000000000, 1.000000000000000000, 0.000000000000000000 ) ) ;
#82772=CARTESIAN_POINT ( 'NONE',  ( -4.800000000000026468, 2.500000000000000000, -4.676537180435978769 ) ) ;
#82773=DIRECTION ( 'NONE',  ( 0.000000000000000000, 0.000000000000000000, -1.000000000000000000 ) ) ;
#82774=DIRECTION ( 'NONE',  ( 0.000000000000000000, 1.000000000000000000, 0.000000000000000000 ) ) ;
#82775=ORIENTED_EDGE ( 'NONE', *, *, #117868, .T. ) ;
#82776=VERTEX_POINT ( 'NONE', #71902 ) ;
#82777=ORIENTED_EDGE ( 'NONE', *, *, #21755, .F. ) ;
#82779=DIRECTION ( 'NONE',  ( 0.000000000000000000, -0.000000000000000000, 1.000000000000000000 ) ) ;
#82780=DIRECTION ( 'NONE',  ( -0.000000000000000000, -1.000000000000000000, -0.000000000000000000 ) ) ;
#82781=DIRECTION ( 'NONE',  ( 0.000000000000000000, 0.000000000000000000, 1.000000000000000000 ) ) ;
#82782=ORIENTED_EDGE ( 'NONE', *, *, #16692, .F. ) ;
#82783=EDGE_CURVE ( 'NONE', #123701, #39867, #103290, .T. ) ;
#82784=FACE_BOUND ( 'NONE', #12683, .T. ) ;
#82785=DIRECTION ( 'NONE',  ( -0.000000000000000000, -1.000000000000000000, -0.000000000000000000 ) ) ;
#82786=LINE ( 'NONE', #114792, #50045 ) ;
#82787=DIRECTION ( 'NONE',  ( 0.000000000000000000, 1.000000000000000000, 0.000000000000000000 ) ) ;
#82788=CIRCLE ( 'NONE', #68086, 0.1000000000000002554 ) ;
#82789=CARTESIAN_POINT ( 'NONE',  ( 11.44999999999991047, 2.500000000000000000, -2.611473670974877592 ) ) ;
#82790=CIRCLE ( 'NONE', #70258, 0.06509327318403745899 ) ;
#82791=CARTESIAN_POINT ( 'NONE',  ( 6.249999999999934275, 12.50000000000000000, -7.188010851410854052 ) ) ;
#82793=LINE ( 'NONE', #2935, #35066 ) ;
#82794=PLANE ( 'NONE',  #128632 ) ;
#82795=DIRECTION ( 'NONE',  ( 0.000000000000000000, -0.000000000000000000, 1.000000000000000000 ) ) ;
#82796=ORIENTED_EDGE ( 'NONE', *, *, #22255, .T. ) ;
#82797=VERTEX_POINT ( 'NONE', #111822 ) ;
#82798=VERTEX_POINT ( 'NONE', #62082 ) ;
#82799=EDGE_LOOP ( 'NONE', ( #39739, #31756, #35167, #42911 ) ) ;
#82800=ORIENTED_EDGE ( 'NONE', *, *, #67736, .F. ) ;
#82801=ORIENTED_EDGE ( 'NONE', *, *, #71579, .T. ) ;
#82802=CIRCLE ( 'NONE', #86884, 0.1000000000000002554 ) ;
#82803=CARTESIAN_POINT ( 'NONE',  ( 5.849999999999934808, 2.500000000000000000, -5.802370205355749988 ) ) ;
#82804=VERTEX_POINT ( 'NONE', #12315 ) ;
#82805=ORIENTED_EDGE ( 'NONE', *, *, #79711, .T. ) ;
#82806=VECTOR ( 'NONE', #106816, 1000.000000000000000 ) ;
#82807=AXIS2_PLACEMENT_3D ( 'NONE', #49, #10506, #11155 ) ;
#82808=ADVANCED_FACE ( 'NONE', ( #59288 ), #47095, .T. ) ;
#82809=PLANE ( 'NONE',  #20387 ) ;
#82810=PLANE ( 'NONE',  #95980 ) ;
#82811=CARTESIAN_POINT ( 'NONE',  ( -0.2000000000000412836, 2.500000000000000000, 4.776537180435972196 ) ) ;
#82812=ORIENTED_EDGE ( 'NONE', *, *, #18699, .T. ) ;
#82813=DIRECTION ( 'NONE',  ( -4.274815082592931898E-19, -0.9999939076577903929, -0.003490651415223739937 ) ) ;
#82814=ORIENTED_EDGE ( 'NONE', *, *, #22842, .T. ) ;
#82815=ORIENTED_EDGE ( 'NONE', *, *, #53430, .T. ) ;
#82816=CARTESIAN_POINT ( 'NONE',  ( 10.84999999999990905, 2.500000000000000000, -7.188010851410854052 ) ) ;
#82817=ADVANCED_FACE ( 'NONE', ( #41584 ), #105668, .T. ) ;
#82818=CARTESIAN_POINT ( 'NONE',  ( 6.449999999999930012, 12.50000000000000000, 1.818653347947321475 ) ) ;
#82819=EDGE_CURVE ( 'NONE', #100751, #62359, #38791, .T. ) ;
#82820=EDGE_CURVE ( 'NONE', #47664, #56350, #19902, .T. ) ;
#82821=EDGE_CURVE ( 'NONE', #97088, #31864, #22051, .T. ) ;
#82822=VECTOR ( 'NONE', #102095, 1000.000000000000000 ) ;
#82823=EDGE_LOOP ( 'NONE', ( #72155, #4952 ) ) ;
#82824=ORIENTED_EDGE ( 'NONE', *, *, #65474, .F. ) ;
#82825=DIRECTION ( 'NONE',  ( -0.000000000000000000, -1.000000000000000000, -0.000000000000000000 ) ) ;
#82826=CARTESIAN_POINT ( 'NONE',  ( -6.050000000000018474, 2.500000000000000000, 2.511473670974873507 ) ) ;
#82827=CARTESIAN_POINT ( 'NONE',  ( -1.250000000000001554, 2.500000000000000000, 2.065063509461097624 ) ) ;
#82828=CIRCLE ( 'NONE', #26385, 0.1000000000000002554 ) ;
#82829=FACE_OUTER_BOUND ( 'NONE', #7120, .T. ) ;
#82830=DIRECTION ( 'NONE',  ( 0.000000000000000000, 1.000000000000000000, 0.000000000000000000 ) ) ;
#82831=AXIS2_PLACEMENT_3D ( 'NONE', #68604, #128854, #8390 ) ;
#82832=EDGE_CURVE ( 'NONE', #93338, #34594, #82593, .T. ) ;
#82833=CIRCLE ( 'NONE', #26393, 0.06509327318403745899 ) ;
#82834=EDGE_LOOP ( 'NONE', ( #46633, #68761 ) ) ;
#82835=DIRECTION ( 'NONE',  ( 0.000000000000000000, 1.000000000000000000, 0.000000000000000000 ) ) ;
#82836=VECTOR ( 'NONE', #80017, 1000.000000000000000 ) ;
#82837=EDGE_CURVE ( 'NONE', #59007, #56480, #68000, .T. ) ;
#82838=EDGE_CURVE ( 'NONE', #75963, #47693, #113975, .T. ) ;
#82839=ORIENTED_EDGE ( 'NONE', *, *, #91738, .T. ) ;
#82840=VECTOR ( 'NONE', #48453, 1000.000000000000000 ) ;
#82841=FACE_OUTER_BOUND ( 'NONE', #93545, .T. ) ;
#82842=EDGE_LOOP ( 'NONE', ( #7942, #91495 ) ) ;
#82843=CARTESIAN_POINT ( 'NONE',  ( 9.549999999999915445, 12.50000000000000000, 6.430097255199259010 ) ) ;
#82844=CARTESIAN_POINT ( 'NONE',  ( 9.999999999999912959, 2.500000000000000000, 3.637306695894644726 ) ) ;
#82845=FACE_OUTER_BOUND ( 'NONE', #101878, .T. ) ;
#82846=DIRECTION ( 'NONE',  ( -0.000000000000000000, 1.000000000000000000, -0.000000000000000000 ) ) ;
#82848=CIRCLE ( 'NONE', #3406, 0.06509327318403745899 ) ;
#82849=CARTESIAN_POINT ( 'NONE',  ( -8.950000000000009948, 2.500000000000000000, -6.841600689897072485 ) ) ;
#82850=AXIS2_PLACEMENT_3D ( 'NONE', #1180, #19527, #9716 ) ;
#82851=VECTOR ( 'NONE', #2106, 1000.000000000000000 ) ;
#82852=DIRECTION ( 'NONE',  ( 0.000000000000000000, 0.000000000000000000, 1.000000000000000000 ) ) ;
#82853=ORIENTED_EDGE ( 'NONE', *, *, #42794, .F. ) ;
#82854=ORIENTED_EDGE ( 'NONE', *, *, #105446, .F. ) ;
#82855=ORIENTED_EDGE ( 'NONE', *, *, #56174, .T. ) ;
#82856=CARTESIAN_POINT ( 'NONE',  ( 17.50000000000000000, 0.9166666666666674068, 10.00000000000000178 ) ) ;
#82857=LINE ( 'NONE', #63199, #13633 ) ;
#82859=DIRECTION ( 'NONE',  ( -0.000000000000000000, 1.000000000000000000, -0.000000000000000000 ) ) ;
#82860=CARTESIAN_POINT ( 'NONE',  ( 8.349999999999923261, 2.500000000000000000, 2.165063509461097713 ) ) ;
#82861=DIRECTION ( 'NONE',  ( -4.274815082592931898E-19, -0.9999939076577903929, -0.003490651415223739937 ) ) ;
#82862=DIRECTION ( 'NONE',  ( 0.000000000000000000, 0.000000000000000000, 1.000000000000000000 ) ) ;
#82863=DIRECTION ( 'NONE',  ( 1.000000000000000000, 0.000000000000000000, 0.000000000000000000 ) ) ;
#82864=ORIENTED_EDGE ( 'NONE', *, *, #129538, .F. ) ;
#82865=DIRECTION ( 'NONE',  ( 0.000000000000000000, 0.000000000000000000, 1.000000000000000000 ) ) ;
#82866=CARTESIAN_POINT ( 'NONE',  ( -3.550000000000030909, 2.500000000000000000, -6.741600689897078169 ) ) ;
#82867=LINE ( 'NONE', #44208, #17195 ) ;
#82868=EDGE_CURVE ( 'NONE', #105143, #87462, #26156, .T. ) ;
#82869=CARTESIAN_POINT ( 'NONE',  ( -14.14999999999998614, 12.50000000000000000, 2.165063509461101265 ) ) ;
#82870=EDGE_LOOP ( 'NONE', ( #120936, #113122, #44733, #122339 ) ) ;
#82871=CARTESIAN_POINT ( 'NONE',  ( -3.550000000000027356, 2.500000000000000000, -2.611473670974877592 ) ) ;
#82872=EDGE_CURVE ( 'NONE', #92109, #66987, #55491, .T. ) ;
#82873=AXIS2_PLACEMENT_3D ( 'NONE', #68125, #89074, #87125 ) ;
#82874=CIRCLE ( 'NONE', #45317, 0.1000000000000002554 ) ;
#82875=EDGE_CURVE ( 'NONE', #103454, #26032, #59626, .T. ) ;
#82876=CARTESIAN_POINT ( 'NONE',  ( -7.100000000000018296, 12.50000000000000000, -4.330127018922201643 ) ) ;
#82877=CARTESIAN_POINT ( 'NONE',  ( -3.350000000000028955, 12.50000000000000000, 2.165063509461097713 ) ) ;
#82878=VERTEX_POINT ( 'NONE', #82127 ) ;
#82879=EDGE_LOOP ( 'NONE', ( #20237, #108631, #8097, #66616 ) ) ;
#82880=EDGE_CURVE ( 'NONE', #126609, #75979, #11558, .T. ) ;
#82881=VECTOR ( 'NONE', #79342, 1000.000000000000000 ) ;
#82882=AXIS2_PLACEMENT_3D ( 'NONE', #102539, #63264, #53460 ) ;
#82883=DIRECTION ( 'NONE',  ( -0.000000000000000000, 1.000000000000000000, -0.000000000000000000 ) ) ;
#82884=ORIENTED_EDGE ( 'NONE', *, *, #90775, .T. ) ;
#82885=ORIENTED_EDGE ( 'NONE', *, *, #49541, .F. ) ;
#82886=LINE ( 'NONE', #73056, #61303 ) ;
#82887=CARTESIAN_POINT ( 'NONE',  ( 14.34999999999989662, 12.50000000000000000, 2.511473670974873507 ) ) ;
#82888=CARTESIAN_POINT ( 'NONE',  ( 10.19999999999991402, 12.50000000000000000, 0.4115034346978109769 ) ) ;
#82889=AXIS2_PLACEMENT_3D ( 'NONE', #48565, #90394, #49866 ) ;
#82890=AXIS2_PLACEMENT_3D ( 'NONE', #30272, #90437, #60992 ) ;
#82891=CARTESIAN_POINT ( 'NONE',  ( -9.400000000000007461, 2.500000000000000000, 3.983716857408420076 ) ) ;
#82892=ORIENTED_EDGE ( 'NONE', *, *, #70358, .T. ) ;
#82893=CARTESIAN_POINT ( 'NONE',  ( -12.29999999999999716, 12.50000000000000000, 0.4115034346978150848 ) ) ;
#82894=DIRECTION ( 'NONE',  ( 0.000000000000000000, 0.000000000000000000, 1.000000000000000000 ) ) ;
#82895=ORIENTED_EDGE ( 'NONE', *, *, #40232, .T. ) ;
#82896=CARTESIAN_POINT ( 'NONE',  ( 16.89179977596970517, 0.9177129796201533019, 5.694535519815870472 ) ) ;
#82897=DIRECTION ( 'NONE',  ( 0.000000000000000000, -0.000000000000000000, 1.000000000000000000 ) ) ;
#82898=VERTEX_POINT ( 'NONE', #69074 ) ;
#82899=ORIENTED_EDGE ( 'NONE', *, *, #128329, .F. ) ;
#82900=EDGE_LOOP ( 'NONE', ( #24556, #101912 ) ) ;
#82901=EDGE_LOOP ( 'NONE', ( #31249, #8484, #92483, #24190 ) ) ;
#82902=DIRECTION ( 'NONE',  ( 0.000000000000000000, 1.000000000000000000, 0.000000000000000000 ) ) ;
#82903=CARTESIAN_POINT ( 'NONE',  ( 13.39053294345161227, 2.500000000000000444, 7.037281288959872150 ) ) ;
#82904=FACE_OUTER_BOUND ( 'NONE', #110238, .T. ) ;
#82905=FACE_BOUND ( 'NONE', #68220, .T. ) ;
#82906=ORIENTED_EDGE ( 'NONE', *, *, #91682, .T. ) ;
#82907=CIRCLE ( 'NONE', #76639, 0.06509327318403745899 ) ;
#82909=DIRECTION ( 'NONE',  ( 0.000000000000000000, 0.000000000000000000, -1.000000000000000000 ) ) ;
#82910=FACE_OUTER_BOUND ( 'NONE', #13575, .T. ) ;
#82911=CIRCLE ( 'NONE', #80854, 0.06509327318403745899 ) ;
#82912=CIRCLE ( 'NONE', #11793, 0.06509327318403745899 ) ;
#82913=ADVANCED_FACE ( 'NONE', ( #40942 ), #128682, .T. ) ;
#82914=FACE_OUTER_BOUND ( 'NONE', #8630, .T. ) ;
#82915=AXIS2_PLACEMENT_3D ( 'NONE', #31919, #40463, #101945 ) ;
#82916=DIRECTION ( 'NONE',  ( -0.000000000000000000, -1.000000000000000000, -0.000000000000000000 ) ) ;
#82917=DIRECTION ( 'NONE',  ( 0.000000000000000000, 1.000000000000000000, 0.000000000000000000 ) ) ;
#82918=CIRCLE ( 'NONE', #3390, 0.09999999999999982514 ) ;
#82919=AXIS2_PLACEMENT_3D ( 'NONE', #3387, #93704, #4021 ) ;
#82920=LINE ( 'NONE', #124767, #82974 ) ;
#82921=ORIENTED_EDGE ( 'NONE', *, *, #121635, .F. ) ;
#82922=EDGE_LOOP ( 'NONE', ( #18684, #113767 ) ) ;
#82923=VERTEX_POINT ( 'NONE', #71660 ) ;
#82924=ORIENTED_EDGE ( 'NONE', *, *, #72621, .T. ) ;
#82925=EDGE_CURVE ( 'NONE', #44661, #24778, #13614, .T. ) ;
#82926=VERTEX_POINT ( 'NONE', #110297 ) ;
#82927=CARTESIAN_POINT ( 'NONE',  ( -4.800000000000024691, 2.500000000000000000, 0.3464101615137735735 ) ) ;
#82928=PLANE ( 'NONE',  #84246 ) ;
#82929=EDGE_LOOP ( 'NONE', ( #92122, #84971, #129386, #40865 ) ) ;
#82930=EDGE_CURVE ( 'NONE', #70218, #85514, #108988, .T. ) ;
#82931=FACE_BOUND ( 'NONE', #98358, .T. ) ;
#82932=DIRECTION ( 'NONE',  ( -0.000000000000000000, -1.000000000000000000, -0.000000000000000000 ) ) ;
#82933=AXIS2_PLACEMENT_3D ( 'NONE', #25988, #105825, #16129 ) ;
#82934=CIRCLE ( 'NONE', #7689, 0.06509327318403745899 ) ;
#82935=VERTEX_POINT ( 'NONE', #11449 ) ;
#82936=DIRECTION ( 'NONE',  ( 0.000000000000000000, 1.000000000000000000, 0.000000000000000000 ) ) ;
#82937=ADVANCED_FACE ( 'NONE', ( #2258 ), #110925, .T. ) ;
#82938=CARTESIAN_POINT ( 'NONE',  ( 2.099999999999948574, 12.50000000000000000, 3.637306695894644726 ) ) ;
#82939=LINE ( 'NONE', #42366, #124863 ) ;
#82940=VERTEX_POINT ( 'NONE', #99200 ) ;
#82941=CARTESIAN_POINT ( 'NONE',  ( -4.550000000000022915, 2.500000000000000000, -2.165063509461101710 ) ) ;
#82942=EDGE_LOOP ( 'NONE', ( #8729, #91063 ) ) ;
#82943=EDGE_LOOP ( 'NONE', ( #36015, #79890 ) ) ;
#82944=VERTEX_POINT ( 'NONE', #80847 ) ;
#82945=FACE_OUTER_BOUND ( 'NONE', #34864, .T. ) ;
#82946=DIRECTION ( 'NONE',  ( -0.000000000000000000, 1.000000000000000000, -0.000000000000000000 ) ) ;
#82947=DIRECTION ( 'NONE',  ( 0.000000000000000000, 0.000000000000000000, -1.000000000000000000 ) ) ;
#82948=EDGE_LOOP ( 'NONE', ( #117011, #74332, #101741, #43785 ) ) ;
#82949=CIRCLE ( 'NONE', #26511, 0.06509327318403745899 ) ;
#82950=DIRECTION ( 'NONE',  ( -0.000000000000000000, 1.000000000000000000, -0.000000000000000000 ) ) ;
#82951=CARTESIAN_POINT ( 'NONE',  ( -8.749999999999975131, 12.50000000000000000, 2.230156782645134950 ) ) ;
#82952=ADVANCED_FACE ( 'NONE', ( #9523 ), #74275, .T. ) ;
#82953=LINE ( 'NONE', #101304, #118399 ) ;
#82954=LINE ( 'NONE', #1787, #3655 ) ;
#82955=VERTEX_POINT ( 'NONE', #14011 ) ;
#82956=CARTESIAN_POINT ( 'NONE',  ( 9.799999999999917222, 2.500000000000000000, 0.4464101615137735513 ) ) ;
#82957=VERTEX_POINT ( 'NONE', #42880 ) ;
#82958=PLANE ( 'NONE',  #120260 ) ;
#82959=ADVANCED_FACE ( 'NONE', ( #84701 ), #65038, .T. ) ;
#82960=CONICAL_SURFACE ( 'NONE', #128946, 0.09999999999999999167, 0.003490658503988666988 ) ;
#82961=EDGE_LOOP ( 'NONE', ( #28875, #70033 ) ) ;
#82962=EDGE_LOOP ( 'NONE', ( #111248, #106304 ) ) ;
#82963=CARTESIAN_POINT ( 'NONE',  ( -11.64999999999999858, 2.500000000000000000, -5.802370205355746435 ) ) ;
#82964=CARTESIAN_POINT ( 'NONE',  ( 2.499999999999948930, 2.500000000000000000, -0.6928203230275541413 ) ) ;
#82965=EDGE_CURVE ( 'NONE', #24381, #125995, #86871, .T. ) ;
#82966=DIRECTION ( 'NONE',  ( 0.000000000000000000, 0.000000000000000000, 1.000000000000000000 ) ) ;
#82967=CARTESIAN_POINT ( 'NONE',  ( 4.999999999999969802, 12.50000000000000000, 4.265033745738159077 ) ) ;
#82968=EDGE_CURVE ( 'NONE', #15244, #58440, #93153, .T. ) ;
#82969=EDGE_CURVE ( 'NONE', #38921, #99960, #72318, .T. ) ;
#82970=CARTESIAN_POINT ( 'NONE',  ( -6.249999999999984901, 12.50000000000000000, -6.495190528383302464 ) ) ;
#82971=EDGE_CURVE ( 'NONE', #118702, #29739, #126603, .T. ) ;
#82973=CIRCLE ( 'NONE', #72509, 0.09999999999999982514 ) ;
#82974=VECTOR ( 'NONE', #54721, 1000.000000000000000 ) ;
#82975=ORIENTED_EDGE ( 'NONE', *, *, #46810, .F. ) ;
#82976=CARTESIAN_POINT ( 'NONE',  ( 2.049999999999950084, 12.50000000000000000, -2.165063509461101710 ) ) ;
#82978=EDGE_CURVE ( 'NONE', #70528, #121075, #76423, .T. ) ;
#82980=ORIENTED_EDGE ( 'NONE', *, *, #116488, .F. ) ;
#82981=VERTEX_POINT ( 'NONE', #124632 ) ;
#82982=EDGE_CURVE ( 'NONE', #89637, #117873, #17917, .T. ) ;
#82983=CONICAL_SURFACE ( 'NONE', #62054, 0.1000000000000000056, 0.003490658503988666988 ) ;
#82984=PLANE ( 'NONE',  #68727 ) ;
#82985=CIRCLE ( 'NONE', #41228, 0.06509327318403745899 ) ;
#82986=AXIS2_PLACEMENT_3D ( 'NONE', #32053, #92226, #11744 ) ;
#82987=ORIENTED_EDGE ( 'NONE', *, *, #60362, .F. ) ;
#82988=DIRECTION ( 'NONE',  ( 0.000000000000000000, 0.000000000000000000, -1.000000000000000000 ) ) ;
#82989=DIRECTION ( 'NONE',  ( -4.274815082592931898E-19, -0.9999939076577903929, -0.003490651415223739937 ) ) ;
#82990=ADVANCED_FACE ( 'NONE', ( #64415 ), #33675, .T. ) ;
#82991=EDGE_CURVE ( 'NONE', #31157, #40264, #112017, .T. ) ;
#82992=DIRECTION ( 'NONE',  ( 0.000000000000000000, 1.000000000000000000, 0.000000000000000000 ) ) ;
#82993=EDGE_LOOP ( 'NONE', ( #10917, #91753, #107466, #42455 ) ) ;
#82994=DIRECTION ( 'NONE',  ( 0.000000000000000000, 0.000000000000000000, 1.000000000000000000 ) ) ;
#82995=DIRECTION ( 'NONE',  ( -0.000000000000000000, -1.000000000000000000, -0.000000000000000000 ) ) ;
#82996=CARTESIAN_POINT ( 'NONE',  ( -5.200000000000020606, 12.50000000000000000, -0.2813168883297408329 ) ) ;
#82997=CARTESIAN_POINT ( 'NONE',  ( -2.900000000000029665, 12.50000000000000000, 4.265033745738159077 ) ) ;
#82998=FACE_OUTER_BOUND ( 'NONE', #90602, .T. ) ;
#82999=EDGE_CURVE ( 'NONE', #37147, #37160, #34337, .T. ) ;
#83000=VERTEX_POINT ( 'NONE', #63787 ) ;
#83001=DIRECTION ( 'NONE',  ( 0.000000000000000000, -0.9999939076577903929, 0.003490651415223739937 ) ) ;
#83002=CARTESIAN_POINT ( 'NONE',  ( 23.85240649353151454, -2.660544618004264006, 4.258220037302151262 ) ) ;
#83003=ORIENTED_EDGE ( 'NONE', *, *, #72640, .F. ) ;
#83004=VERTEX_POINT ( 'NONE', #34984 ) ;
#83006=DIRECTION ( 'NONE',  ( 0.000000000000000000, 0.000000000000000000, 1.000000000000000000 ) ) ;
#83007=AXIS2_PLACEMENT_3D ( 'NONE', #95987, #86804, #114330 ) ;
#83008=CARTESIAN_POINT ( 'NONE',  ( -12.09999999999999609, 2.500000000000000000, -0.6928203230275501445 ) ) ;
#83009=AXIS2_PLACEMENT_3D ( 'NONE', #43203, #90993, #101464 ) ;
#83010=CARTESIAN_POINT ( 'NONE',  ( 8.549999999999918998, 12.50000000000000000, 6.841600689897072485 ) ) ;
#83011=CONICAL_SURFACE ( 'NONE', #34990, 0.1000000000000000056, 0.003490658503988666988 ) ;
#83012=DIRECTION ( 'NONE',  ( 0.000000000000000000, 0.000000000000000000, 1.000000000000000000 ) ) ;
#83013=DIRECTION ( 'NONE',  ( 0.000000000000000000, 0.000000000000000000, 1.000000000000000000 ) ) ;
#83014=AXIS2_PLACEMENT_3D ( 'NONE', #4790, #4143, #114120 ) ;
#83015=DIRECTION ( 'NONE',  ( -0.000000000000000000, 1.000000000000000000, -0.000000000000000000 ) ) ;
#83016=DIRECTION ( 'NONE',  ( 0.000000000000000000, 0.000000000000000000, -1.000000000000000000 ) ) ;
#83017=DIRECTION ( 'NONE',  ( -0.000000000000000000, -1.000000000000000000, -0.000000000000000000 ) ) ;
#83018=VECTOR ( 'NONE', #13527, 1000.000000000000000 ) ;
#83019=VECTOR ( 'NONE', #6911, 1000.000000000000000 ) ;
#83020=CARTESIAN_POINT ( 'NONE',  ( 0.8499999999999550138, 2.500000000000000000, -5.902370205355750521 ) ) ;
#83021=ORIENTED_EDGE ( 'NONE', *, *, #40064, .F. ) ;
#83022=ORIENTED_EDGE ( 'NONE', *, *, #24267, .T. ) ;
#83023=AXIS2_PLACEMENT_3D ( 'NONE', #94287, #104739, #102810 ) ;
#83024=ORIENTED_EDGE ( 'NONE', *, *, #46870, .T. ) ;
#83025=ORIENTED_EDGE ( 'NONE', *, *, #42020, .T. ) ;
#83026=DIRECTION ( 'NONE',  ( 0.000000000000000000, 0.000000000000000000, 1.000000000000000000 ) ) ;
#83027=CARTESIAN_POINT ( 'NONE',  ( -8.950000000000008171, 2.500000000000000000, 1.818653347947321475 ) ) ;
#83028=VECTOR ( 'NONE', #110106, 1000.000000000000000 ) ;
#83029=ORIENTED_EDGE ( 'NONE', *, *, #88429, .T. ) ;
#83030=CARTESIAN_POINT ( 'NONE',  ( 4.599999999999936584, 2.500000000000000000, 3.637306695894644726 ) ) ;
#83031=EDGE_CURVE ( 'NONE', #92919, #37333, #45122, .T. ) ;
#83032=AXIS2_PLACEMENT_3D ( 'NONE', #46761, #114206, #46107 ) ;
#83033=AXIS2_PLACEMENT_3D ( 'NONE', #120925, #36747, #78609 ) ;
#83034=ADVANCED_FACE ( 'NONE', ( #74891 ), #36718, .T. ) ;
#83035=CARTESIAN_POINT ( 'NONE',  ( -0.8000000000000376810, 2.500000000000000000, -4.430127018922202176 ) ) ;
#83036=CARTESIAN_POINT ( 'NONE',  ( -3.300000000000027800, 12.50000000000000000, -0.06509327318403970719 ) ) ;
#83037=EDGE_LOOP ( 'NONE', ( #125260, #61522, #128512, #95160 ) ) ;
#83038=CARTESIAN_POINT ( 'NONE',  ( -4.150000000000024336, 12.50000000000000000, -2.165063509461101710 ) ) ;
#83039=CARTESIAN_POINT ( 'NONE',  ( 2.899999999999943956, 12.50000000000000000, 4.330127018922196314 ) ) ;
#83040=ORIENTED_EDGE ( 'NONE', *, *, #79411, .T. ) ;
#83042=VERTEX_POINT ( 'NONE', #103711 ) ;
#83043=ORIENTED_EDGE ( 'NONE', *, *, #51888, .F. ) ;
#83044=CARTESIAN_POINT ( 'NONE',  ( -14.79999999999998472, 12.50000000000000000, 0.2813168883297384459 ) ) ;
#83045=AXIS2_PLACEMENT_3D ( 'NONE', #113044, #124156, #23365 ) ;
#83046=FACE_OUTER_BOUND ( 'NONE', #69165, .T. ) ;
#83047=CARTESIAN_POINT ( 'NONE',  ( 5.399999999999936406, 12.50000000000000000, -3.637306695894650055 ) ) ;
#83048=DIRECTION ( 'NONE',  ( 0.000000000000000000, 0.000000000000000000, 1.000000000000000000 ) ) ;
#83049=ORIENTED_EDGE ( 'NONE', *, *, #66839, .F. ) ;
#83050=CARTESIAN_POINT ( 'NONE',  ( -11.89999999999999680, 12.50000000000000000, -3.918623584224386391 ) ) ;
#83051=VERTEX_POINT ( 'NONE', #15294 ) ;
#83053=CARTESIAN_POINT ( 'NONE',  ( 8.497934422427476875, -1.500000000000508038, -9.526046680185665139 ) ) ;
#83054=DIRECTION ( 'NONE',  ( 0.000000000000000000, -0.9999939076577903929, 0.003490651415223739937 ) ) ;
#83055=FACE_OUTER_BOUND ( 'NONE', #49480, .T. ) ;
#83056=VERTEX_POINT ( 'NONE', #12721 ) ;
#83057=CONICAL_SURFACE ( 'NONE', #95568, 0.1000000000000002554, 0.003490658503988666988 ) ;
#83058=CIRCLE ( 'NONE', #76787, 0.09999999999999982514 ) ;
#83059=VERTEX_POINT ( 'NONE', #104964 ) ;
#83060=VERTEX_POINT ( 'NONE', #13378 ) ;
#83061=DIRECTION ( 'NONE',  ( 0.000000000000000000, 0.000000000000000000, 1.000000000000000000 ) ) ;
#83062=PLANE ( 'NONE',  #64450 ) ;
#83063=CARTESIAN_POINT ( 'NONE',  ( 9.349999999999916156, 2.500000000000000000, -1.918653347947326004 ) ) ;
#83064=FACE_BOUND ( 'NONE', #59683, .T. ) ;
#83065=DIRECTION ( 'NONE',  ( -0.000000000000000000, -1.000000000000000000, -0.000000000000000000 ) ) ;
#83066=DIRECTION ( 'NONE',  ( 0.000000000000000000, 1.000000000000000000, 0.000000000000000000 ) ) ;
#83068=CIRCLE ( 'NONE', #93521, 0.06509327318403743123 ) ;
#83069=LINE ( 'NONE', #122987, #127298 ) ;
#83070=EDGE_CURVE ( 'NONE', #76977, #80050, #53960, .T. ) ;
#83071=CIRCLE ( 'NONE', #76800, 0.06509327318403745899 ) ;
#83072=FACE_OUTER_BOUND ( 'NONE', #51094, .T. ) ;
#83073=CARTESIAN_POINT ( 'NONE',  ( 1.649999999999950617, 2.500000000000000000, -2.165063509461101710 ) ) ;
#83074=FACE_OUTER_BOUND ( 'NONE', #19599, .T. ) ;
#83075=ORIENTED_EDGE ( 'NONE', *, *, #60865, .F. ) ;
#83076=AXIS2_PLACEMENT_3D ( 'NONE', #52114, #1064, #80287 ) ;
#83077=AXIS2_PLACEMENT_3D ( 'NONE', #83719, #14305, #75807 ) ;
#83078=AXIS2_PLACEMENT_3D ( 'NONE', #76812, #116717, #27064 ) ;
#83079=DIRECTION ( 'NONE',  ( -0.000000000000000000, 1.000000000000000000, -0.000000000000000000 ) ) ;
#83080=ORIENTED_EDGE ( 'NONE', *, *, #125839, .F. ) ;
#83081=VERTEX_POINT ( 'NONE', #95172 ) ;
#83082=EDGE_CURVE ( 'NONE', #78931, #10631, #72958, .T. ) ;
#83083=CARTESIAN_POINT ( 'NONE',  ( 7.699999999999925571, 12.50000000000000000, 3.983716857408420076 ) ) ;
#83084=CARTESIAN_POINT ( 'NONE',  ( 3.749999999999978684, 12.50000000000000000, -2.165063509461101710 ) ) ;
#83085=EDGE_CURVE ( 'NONE', #97899, #73263, #2933, .T. ) ;
#83086=FACE_BOUND ( 'NONE', #98690, .T. ) ;
#83087=DIRECTION ( 'NONE',  ( 0.000000000000000000, 1.000000000000000000, 0.000000000000000000 ) ) ;
#83088=AXIS2_PLACEMENT_3D ( 'NONE', #1624, #41586, #121403 ) ;
#83089=VERTEX_POINT ( 'NONE', #103045 ) ;
#83090=CARTESIAN_POINT ( 'NONE',  ( 65.40459994261938448, 3.824478557803584700, 5.306485876514984490 ) ) ;
#83091=EDGE_CURVE ( 'NONE', #38337, #69557, #103616, .T. ) ;
#83092=CARTESIAN_POINT ( 'NONE',  ( -11.69999999999999574, 2.500000000000000000, 4.430127018922196847 ) ) ;
#83093=CIRCLE ( 'NONE', #43394, 0.06509327318403745899 ) ;
#83094=ORIENTED_EDGE ( 'NONE', *, *, #28112, .T. ) ;
#83095=DIRECTION ( 'NONE',  ( 0.000000000000000000, -0.000000000000000000, 1.000000000000000000 ) ) ;
#83096=AXIS2_PLACEMENT_3D ( 'NONE', #87775, #50439, #19032 ) ;
#83097=DIRECTION ( 'NONE',  ( 0.000000000000000000, -0.000000000000000000, 1.000000000000000000 ) ) ;
#83098=AXIS2_PLACEMENT_3D ( 'NONE', #67719, #38954, #128620 ) ;
#83099=EDGE_LOOP ( 'NONE', ( #4059, #49697 ) ) ;
#83100=PLANE ( 'NONE',  #115446 ) ;
#83101=CARTESIAN_POINT ( 'NONE',  ( -11.64999999999999680, 12.50000000000000000, -6.495190528383298911 ) ) ;
#83102=AXIS2_PLACEMENT_3D ( 'NONE', #34339, #3565, #33676 ) ;
#83103=AXIS2_PLACEMENT_3D ( 'NONE', #78927, #30476, #70378 ) ;
#83104=ORIENTED_EDGE ( 'NONE', *, *, #5892, .T. ) ;
#83105=CIRCLE ( 'NONE', #127116, 0.1000000000000000472 ) ;
#83106=DIRECTION ( 'NONE',  ( 0.000000000000000000, 0.000000000000000000, 1.000000000000000000 ) ) ;
#83107=DIRECTION ( 'NONE',  ( 0.000000000000000000, 0.000000000000000000, -1.000000000000000000 ) ) ;
#83108=CARTESIAN_POINT ( 'NONE',  ( -8.950000000000009948, 12.50000000000000000, -6.841600689897072485 ) ) ;
#83109=VERTEX_POINT ( 'NONE', #115419 ) ;
#83110=EDGE_LOOP ( 'NONE', ( #38712, #90417, #9067, #48801 ) ) ;
#83111=CIRCLE ( 'NONE', #32955, 0.1000000000000002554 ) ;
#83113=EDGE_LOOP ( 'NONE', ( #82114, #89558 ) ) ;
#83114=DIRECTION ( 'NONE',  ( 0.000000000000000000, 1.000000000000000000, 0.000000000000000000 ) ) ;
#83115=CARTESIAN_POINT ( 'NONE',  ( 13.94999999999989804, 12.50000000000000000, 1.818653347947321475 ) ) ;
#83116=ADVANCED_FACE ( 'NONE', ( #125900 ), #75513, .T. ) ;
#83117=CIRCLE ( 'NONE', #112459, 0.06509327318403745899 ) ;
#83118=VECTOR ( 'NONE', #32576, 1000.000000000000000 ) ;
#83119=ORIENTED_EDGE ( 'NONE', *, *, #85053, .F. ) ;
#83120=DIRECTION ( 'NONE',  ( 0.000000000000000000, 0.000000000000000000, 1.000000000000000000 ) ) ;
#83121=PLANE ( 'NONE',  #20537 ) ;
#83122=DIRECTION ( 'NONE',  ( -4.274815082592931898E-19, -0.9999939076577903929, -0.003490651415223739937 ) ) ;
#83123=DIRECTION ( 'NONE',  ( -4.274815082592931898E-19, -0.9999939076577903929, -0.003490651415223739937 ) ) ;
#83125=EDGE_CURVE ( 'NONE', #16607, #46996, #87532, .T. ) ;
#83126=FACE_OUTER_BOUND ( 'NONE', #100485, .T. ) ;
#83127=EDGE_CURVE ( 'NONE', #102950, #111853, #106907, .T. ) ;
#83128=EDGE_LOOP ( 'NONE', ( #50994, #69739, #81957, #60105 ) ) ;
#83129=EDGE_LOOP ( 'NONE', ( #55806, #94367 ) ) ;
#83130=CARTESIAN_POINT ( 'NONE',  ( -1.700000000000034817, 12.50000000000000000, -4.395220292106239768 ) ) ;
#83131=ORIENTED_EDGE ( 'NONE', *, *, #58004, .F. ) ;
#83132=PLANE ( 'NONE',  #89001 ) ;
#83133=EDGE_CURVE ( 'NONE', #19378, #123253, #53441, .T. ) ;
#83134=ORIENTED_EDGE ( 'NONE', *, *, #110163, .T. ) ;
#83135=ORIENTED_EDGE ( 'NONE', *, *, #913, .F. ) ;
#83136=EDGE_CURVE ( 'NONE', #18239, #122843, #6128, .T. ) ;
#83137=ORIENTED_EDGE ( 'NONE', *, *, #46600, .T. ) ;
#83138=ADVANCED_FACE ( 'NONE', ( #106277 ), #78585, .T. ) ;
#83139=CIRCLE ( 'NONE', #30824, 0.1000000000000002554 ) ;
#83140=CARTESIAN_POINT ( 'NONE',  ( -7.900000000000014566, 2.500000000000000000, -4.230127018922201998 ) ) ;
#83141=DIRECTION ( 'NONE',  ( 0.000000000000000000, 0.000000000000000000, -1.000000000000000000 ) ) ;
#83142=PLANE ( 'NONE',  #45629 ) ;
#83144=EDGE_CURVE ( 'NONE', #18181, #103538, #79652, .T. ) ;
#83145=DIRECTION ( 'NONE',  ( 0.000000000000000000, 1.000000000000000000, 0.000000000000000000 ) ) ;
#83146=DIRECTION ( 'NONE',  ( 0.000000000000000000, 1.000000000000000000, 0.000000000000000000 ) ) ;
#83149=CARTESIAN_POINT ( 'NONE',  ( 6.449999999999930012, 2.500000000000000000, -1.818653347947326138 ) ) ;
#83150=CARTESIAN_POINT ( 'NONE',  ( -11.89999999999999680, 12.50000000000000000, 0.3464101615137776813 ) ) ;
#83151=ADVANCED_FACE ( 'NONE', ( #17888 ), #96439, .T. ) ;
#83152=CIRCLE ( 'NONE', #70515, 0.06509327318403745899 ) ;
#83153=ORIENTED_EDGE ( 'NONE', *, *, #111325, .T. ) ;
#83154=CIRCLE ( 'NONE', #45585, 0.1000000000000002554 ) ;
#83155=DIRECTION ( 'NONE',  ( 0.000000000000000000, -0.000000000000000000, 1.000000000000000000 ) ) ;
#83156=ORIENTED_EDGE ( 'NONE', *, *, #79971, .F. ) ;
#83157=ORIENTED_EDGE ( 'NONE', *, *, #3712, .T. ) ;
#83158=DIRECTION ( 'NONE',  ( -0.000000000000000000, 1.000000000000000000, -0.000000000000000000 ) ) ;
#83159=DIRECTION ( 'NONE',  ( 0.000000000000000000, 0.000000000000000000, 1.000000000000000000 ) ) ;
#83160=DIRECTION ( 'NONE',  ( -0.000000000000000000, 1.000000000000000000, -0.000000000000000000 ) ) ;
#83161=CIRCLE ( 'NONE', #26715, 0.06509327318403745899 ) ;
#83163=VECTOR ( 'NONE', #62362, 1000.000000000000000 ) ;
#83164=DIRECTION ( 'NONE',  ( -4.274815082592931898E-19, -0.9999939076577903929, -0.003490651415223739937 ) ) ;
#83165=LINE ( 'NONE', #22949, #105483 ) ;
#83166=CARTESIAN_POINT ( 'NONE',  ( 15.39999999999989200, 12.50000000000000000, 0.6928203230275494784 ) ) ;
#83167=VERTEX_POINT ( 'NONE', #6751 ) ;
#83168=CARTESIAN_POINT ( 'NONE',  ( -3.350000000000028955, 2.500000000000000000, 7.088010851410848190 ) ) ;
#83170=AXIS2_PLACEMENT_3D ( 'NONE', #1305, #19666, #658 ) ;
#83171=EDGE_LOOP ( 'NONE', ( #55434, #48042, #8793, #21068 ) ) ;
#83172=VERTEX_POINT ( 'NONE', #46713 ) ;
#83173=AXIS2_PLACEMENT_3D ( 'NONE', #107635, #47433, #89283 ) ;
#83174=ORIENTED_EDGE ( 'NONE', *, *, #117951, .T. ) ;
#83175=DIRECTION ( 'NONE',  ( 0.000000000000000000, 0.000000000000000000, 1.000000000000000000 ) ) ;
#83176=CARTESIAN_POINT ( 'NONE',  ( -10.80000000000000071, 12.50000000000000000, 4.265033745738159077 ) ) ;
#83177=VECTOR ( 'NONE', #123, 1000.000000000000000 ) ;
#83178=DIRECTION ( 'NONE',  ( -0.000000000000000000, 1.000000000000000000, -0.000000000000000000 ) ) ;
#83179=EDGE_CURVE ( 'NONE', #42996, #14604, #8694, .T. ) ;
#83180=CARTESIAN_POINT ( 'NONE',  ( 2.499999999999983569, 2.500000000000000000, -4.330127018922201643 ) ) ;
#83182=PLANE ( 'NONE',  #99442 ) ;
#83183=EDGE_LOOP ( 'NONE', ( #50492, #93917 ) ) ;
#83184=PLANE ( 'NONE',  #1393 ) ;
#83185=DIRECTION ( 'NONE',  ( -0.000000000000000000, -1.000000000000000000, -0.000000000000000000 ) ) ;
#83186=CARTESIAN_POINT ( 'NONE',  ( 4.349999999999941025, 2.500000000000000000, -6.248780366869526759 ) ) ;
#83187=CIRCLE ( 'NONE', #16339, 0.1000000000000002554 ) ;
#83188=VECTOR ( 'NONE', #54947, 1000.000000000000000 ) ;
#83189=CARTESIAN_POINT ( 'NONE',  ( 0.7999999999999612976, 12.50000000000000000, -0.06509327318403752838 ) ) ;
#83190=EDGE_CURVE ( 'NONE', #98077, #104184, #57640, .T. ) ;
#83191=ORIENTED_EDGE ( 'NONE', *, *, #44977, .F. ) ;
#83192=CIRCLE ( 'NONE', #28811, 0.06509327318403741736 ) ;
#83193=EDGE_LOOP ( 'NONE', ( #102692, #104226 ) ) ;
#83194=ORIENTED_EDGE ( 'NONE', *, *, #4358, .T. ) ;
#83195=DIRECTION ( 'NONE',  ( -0.000000000000000000, 1.000000000000000000, -0.000000000000000000 ) ) ;
#83196=AXIS2_PLACEMENT_3D ( 'NONE', #66344, #36906, #66974 ) ;
#83197=AXIS2_PLACEMENT_3D ( 'NONE', #6755, #35617, #76183 ) ;
#83198=CARTESIAN_POINT ( 'NONE',  ( 3.349999999999945466, 12.50000000000000000, -2.922977105672691422 ) ) ;
#83199=DIRECTION ( 'NONE',  ( 0.000000000000000000, 0.000000000000000000, -1.000000000000000000 ) ) ;
#83200=ORIENTED_EDGE ( 'NONE', *, *, #16369, .T. ) ;
#83201=DIRECTION ( 'NONE',  ( 0.000000000000000000, -0.9999939076577903929, 0.003490651415223739937 ) ) ;
#83202=CARTESIAN_POINT ( 'NONE',  ( 1.249999999999954259, 2.500000000000000000, -7.188010851410854052 ) ) ;
#83203=AXIS2_PLACEMENT_3D ( 'NONE', #64606, #26620, #46250 ) ;
#83204=CARTESIAN_POINT ( 'NONE',  ( -6.700000000000016165, 12.50000000000000000, 4.265033745738159077 ) ) ;
#83205=DIRECTION ( 'NONE',  ( 0.000000000000000000, 1.000000000000000000, 0.000000000000000000 ) ) ;
#83206=CIRCLE ( 'NONE', #22586, 0.1000000000000002554 ) ;
#83207=CIRCLE ( 'NONE', #45555, 0.06509327318403741736 ) ;
#83208=CARTESIAN_POINT ( 'NONE',  ( 1.649999999999950617, 2.500000000000000000, -2.065063509461102065 ) ) ;
#83209=VERTEX_POINT ( 'NONE', #65703 ) ;
#83210=EDGE_LOOP ( 'NONE', ( #85530, #24074, #38417, #38199 ) ) ;
#83211=CARTESIAN_POINT ( 'NONE',  ( 10.19999999999991047, 2.500000000000000000, -3.983716857408426293 ) ) ;
#83212=DIRECTION ( 'NONE',  ( -0.000000000000000000, -1.000000000000000000, -0.000000000000000000 ) ) ;
#83213=DIRECTION ( 'NONE',  ( -0.000000000000000000, 1.000000000000000000, -0.000000000000000000 ) ) ;
#83214=CARTESIAN_POINT ( 'NONE',  ( 7.049999999999930544, 2.500000000000000000, -6.495190528383302464 ) ) ;
#83215=FACE_OUTER_BOUND ( 'NONE', #100339, .T. ) ;
#83216=EDGE_CURVE ( 'NONE', #33924, #103702, #15855, .T. ) ;
#83217=ORIENTED_EDGE ( 'NONE', *, *, #116818, .T. ) ;
#83218=ORIENTED_EDGE ( 'NONE', *, *, #79715, .T. ) ;
#83219=CARTESIAN_POINT ( 'NONE',  ( 5.199999999999937117, 2.500000000000000000, -4.676537180435978769 ) ) ;
#83220=DIRECTION ( 'NONE',  ( 0.000000000000000000, 1.000000000000000000, 0.000000000000000000 ) ) ;
#83221=DIRECTION ( 'NONE',  ( 0.000000000000000000, 0.000000000000000000, 1.000000000000000000 ) ) ;
#83222=DIRECTION ( 'NONE',  ( 0.000000000000000000, 0.000000000000000000, 1.000000000000000000 ) ) ;
#83224=ORIENTED_EDGE ( 'NONE', *, *, #15513, .F. ) ;
#83225=EDGE_CURVE ( 'NONE', #56742, #114427, #47176, .T. ) ;
#83226=FACE_OUTER_BOUND ( 'NONE', #52622, .T. ) ;
#83227=DIRECTION ( 'NONE',  ( -0.000000000000000000, 1.000000000000000000, -0.000000000000000000 ) ) ;
#83228=AXIS2_PLACEMENT_3D ( 'NONE', #50421, #100794, #90326 ) ;
#83229=ORIENTED_EDGE ( 'NONE', *, *, #25325, .T. ) ;
#83230=CIRCLE ( 'NONE', #104150, 0.06509327318403745899 ) ;
#83232=CARTESIAN_POINT ( 'NONE',  ( 5.399999999999931966, 2.500000000000000000, 4.230127018922196669 ) ) ;
#83233=ADVANCED_FACE ( 'NONE', ( #78113 ), #35613, .T. ) ;
#83234=EDGE_LOOP ( 'NONE', ( #63465, #111012, #83829, #35937 ) ) ;
#83235=DIRECTION ( 'NONE',  ( 0.000000000000000000, 1.000000000000000000, 0.000000000000000000 ) ) ;
#83236=VECTOR ( 'NONE', #80726, 1000.000000000000000 ) ;
#83237=AXIS2_PLACEMENT_3D ( 'NONE', #65475, #105415, #5895 ) ;
#83238=ORIENTED_EDGE ( 'NONE', *, *, #46770, .F. ) ;
#83239=PLANE ( 'NONE',  #102934 ) ;
#83240=FACE_OUTER_BOUND ( 'NONE', #19453, .T. ) ;
#83241=EDGE_CURVE ( 'NONE', #127171, #13735, #105641, .T. ) ;
#83242=ORIENTED_EDGE ( 'NONE', *, *, #116844, .T. ) ;
#83243=ORIENTED_EDGE ( 'NONE', *, *, #118872, .F. ) ;
#83244=EDGE_CURVE ( 'NONE', #74924, #48671, #105754, .T. ) ;
#83246=DIRECTION ( 'NONE',  ( -0.000000000000000000, -1.000000000000000000, -0.000000000000000000 ) ) ;
#83247=AXIS2_PLACEMENT_3D ( 'NONE', #113804, #116363, #45712 ) ;
#83248=CARTESIAN_POINT ( 'NONE',  ( 11.84999999999990372, 2.500000000000000000, 1.918653347947321564 ) ) ;
#83250=AXIS2_PLACEMENT_3D ( 'NONE', #119106, #77876, #20261 ) ;
#83251=FACE_OUTER_BOUND ( 'NONE', #101208, .T. ) ;
#83252=FACE_OUTER_BOUND ( 'NONE', #85642, .T. ) ;
#83253=DIRECTION ( 'NONE',  ( 0.000000000000000000, 1.000000000000000000, 0.000000000000000000 ) ) ;
#83254=DIRECTION ( 'NONE',  ( -0.000000000000000000, 1.000000000000000000, -0.000000000000000000 ) ) ;
#83255=VECTOR ( 'NONE', #38533, 1000.000000000000000 ) ;
#83256=ORIENTED_EDGE ( 'NONE', *, *, #30653, .F. ) ;
#83257=ORIENTED_EDGE ( 'NONE', *, *, #68880, .T. ) ;
#83258=DIRECTION ( 'NONE',  ( -0.000000000000000000, 1.000000000000000000, -0.000000000000000000 ) ) ;
#83259=VERTEX_POINT ( 'NONE', #37550 ) ;
#83261=DIRECTION ( 'NONE',  ( -0.000000000000000000, -1.000000000000000000, -0.000000000000000000 ) ) ;
#83262=AXIS2_PLACEMENT_3D ( 'NONE', #92493, #102957, #111490 ) ;
#83263=CARTESIAN_POINT ( 'NONE',  ( -2.900000000000029665, 2.500000000000000000, 4.230127018922196669 ) ) ;
#83264=VERTEX_POINT ( 'NONE', #77458 ) ;
#83265=VERTEX_POINT ( 'NONE', #72175 ) ;
#83266=LINE ( 'NONE', #103549, #108048 ) ;
#83267=VERTEX_POINT ( 'NONE', #49966 ) ;
#83268=DIRECTION ( 'NONE',  ( 0.000000000000000000, 0.000000000000000000, 1.000000000000000000 ) ) ;
#83269=LINE ( 'NONE', #32249, #54033 ) ;
#83270=FACE_OUTER_BOUND ( 'NONE', #1459, .T. ) ;
#83271=VECTOR ( 'NONE', #100690, 1000.000000000000000 ) ;
#83272=CARTESIAN_POINT ( 'NONE',  ( 1.699999999999950218, 12.50000000000000000, 4.395220292106234439 ) ) ;
#83273=LINE ( 'NONE', #115262, #38873 ) ;
#83274=DIRECTION ( 'NONE',  ( 0.000000000000000000, 0.000000000000000000, 1.000000000000000000 ) ) ;
#83275=DIRECTION ( 'NONE',  ( 0.000000000000000000, -0.000000000000000000, 1.000000000000000000 ) ) ;
#83276=DIRECTION ( 'NONE',  ( 0.000000000000000000, 0.000000000000000000, 1.000000000000000000 ) ) ;
#83277=DIRECTION ( 'NONE',  ( 0.000000000000000000, 0.000000000000000000, 1.000000000000000000 ) ) ;
#83278=CARTESIAN_POINT ( 'NONE',  ( 6.249999999999965361, 12.50000000000000000, 2.099970236277060032 ) ) ;
#83279=AXIS2_PLACEMENT_3D ( 'NONE', #104057, #14366, #116439 ) ;
#83280=DIRECTION ( 'NONE',  ( 0.000000000000000000, 0.000000000000000000, 1.000000000000000000 ) ) ;
#83281=ADVANCED_FACE ( 'NONE', ( #177 ), #97342, .T. ) ;
#83282=VERTEX_POINT ( 'NONE', #52513 ) ;
#83283=CIRCLE ( 'NONE', #87457, 0.09999999999999982514 ) ;
#83284=ORIENTED_EDGE ( 'NONE', *, *, #16460, .F. ) ;
#83285=ORIENTED_EDGE ( 'NONE', *, *, #33156, .F. ) ;
#83286=PLANE ( 'NONE',  #128589 ) ;
#83287=ORIENTED_EDGE ( 'NONE', *, *, #95097, .T. ) ;
#83288=DIRECTION ( 'NONE',  ( 0.000000000000000000, -0.000000000000000000, 1.000000000000000000 ) ) ;
#83289=EDGE_CURVE ( 'NONE', #120080, #71030, #19989, .T. ) ;
#83290=ORIENTED_EDGE ( 'NONE', *, *, #101860, .T. ) ;
#83291=ORIENTED_EDGE ( 'NONE', *, *, #18812, .F. ) ;
#83292=ORIENTED_EDGE ( 'NONE', *, *, #62702, .F. ) ;
#83293=CIRCLE ( 'NONE', #81228, 0.06509327318403745899 ) ;
#83294=ADVANCED_FACE ( 'NONE', ( #51887 ), #32261, .T. ) ;
#83295=DIRECTION ( 'NONE',  ( 0.000000000000000000, 0.000000000000000000, -1.000000000000000000 ) ) ;
#83296=EDGE_CURVE ( 'NONE', #20888, #85559, #21785, .T. ) ;
#83297=DIRECTION ( 'NONE',  ( -0.000000000000000000, 1.000000000000000000, -0.000000000000000000 ) ) ;
#83299=EDGE_CURVE ( 'NONE', #38578, #65715, #9606, .T. ) ;
#83300=DIRECTION ( 'NONE',  ( 0.000000000000000000, 1.000000000000000000, 0.000000000000000000 ) ) ;
#83301=DIRECTION ( 'NONE',  ( 0.000000000000000000, 0.000000000000000000, -1.000000000000000000 ) ) ;
#83302=DIRECTION ( 'NONE',  ( 0.000000000000000000, 0.000000000000000000, 1.000000000000000000 ) ) ;
#83303=VERTEX_POINT ( 'NONE', #81348 ) ;
#83304=DIRECTION ( 'NONE',  ( 0.000000000000000000, 0.000000000000000000, 1.000000000000000000 ) ) ;
#83305=EDGE_CURVE ( 'NONE', #73593, #66462, #82788, .T. ) ;
#83306=EDGE_LOOP ( 'NONE', ( #3615, #109746 ) ) ;
#83307=VECTOR ( 'NONE', #100269, 1000.000000000000000 ) ;
#83308=EDGE_CURVE ( 'NONE', #89740, #47635, #90493, .T. ) ;
#83309=ORIENTED_EDGE ( 'NONE', *, *, #90792, .F. ) ;
#83310=EDGE_LOOP ( 'NONE', ( #120534, #4916, #7150, #107714 ) ) ;
#83311=DIRECTION ( 'NONE',  ( 0.000000000000000000, -0.9999939076577903929, 0.003490651415223739937 ) ) ;
#83313=ORIENTED_EDGE ( 'NONE', *, *, #72630, .F. ) ;
#83314=ORIENTED_EDGE ( 'NONE', *, *, #31111, .F. ) ;
#83316=DIRECTION ( 'NONE',  ( 0.000000000000000000, -0.000000000000000000, 1.000000000000000000 ) ) ;
#83317=CARTESIAN_POINT ( 'NONE',  ( -13.34999999999999076, 2.500000000000000000, -2.265063509461099578 ) ) ;
#83318=CARTESIAN_POINT ( 'NONE',  ( 6.649999999999931966, 2.500000000000000000, -5.802370205355749988 ) ) ;
#83319=CARTESIAN_POINT ( 'NONE',  ( -12.49999999999999289, 12.50000000000000000, -0.6928203230275500335 ) ) ;
#83320=PLANE ( 'NONE',  #4862 ) ;
#83321=CIRCLE ( 'NONE', #51927, 0.1000000000000002554 ) ;
#83322=EDGE_CURVE ( 'NONE', #115754, #21052, #26344, .T. ) ;
#83323=CARTESIAN_POINT ( 'NONE',  ( 0.8499999999999557909, 12.50000000000000000, -7.188010851410854052 ) ) ;
#83324=ORIENTED_EDGE ( 'NONE', *, *, #38205, .F. ) ;
#83325=CONICAL_SURFACE ( 'NONE', #72850, 0.1000000000000002554, 0.003490658503988666988 ) ;
#83326=LINE ( 'NONE', #33580, #50589 ) ;
#83327=VECTOR ( 'NONE', #24239, 1000.000000000000000 ) ;
#83328=ORIENTED_EDGE ( 'NONE', *, *, #109890, .F. ) ;
#83329=DIRECTION ( 'NONE',  ( 0.000000000000000000, 0.000000000000000000, -1.000000000000000000 ) ) ;
#83330=AXIS2_PLACEMENT_3D ( 'NONE', #88929, #57538, #99400 ) ;
#83332=ORIENTED_EDGE ( 'NONE', *, *, #68211, .F. ) ;
#83333=AXIS2_PLACEMENT_3D ( 'NONE', #110941, #71680, #24996 ) ;
#83334=CARTESIAN_POINT ( 'NONE',  ( -6.250000000000019540, 12.50000000000000000, -2.857883832488653741 ) ) ;
#83335=CARTESIAN_POINT ( 'NONE',  ( 12.29999999999990656, 2.500000000000000000, -4.676537180435977881 ) ) ;
#83336=CIRCLE ( 'NONE', #60355, 0.1000000000000000056 ) ;
#83337=AXIS2_PLACEMENT_3D ( 'NONE', #64832, #115872, #113946 ) ;
#83338=VECTOR ( 'NONE', #102268, 1000.000000000000000 ) ;
#83339=CARTESIAN_POINT ( 'NONE',  ( -10.84999999999999964, 2.500000000000000000, 2.857883832488649301 ) ) ;
#83340=ORIENTED_EDGE ( 'NONE', *, *, #111341, .T. ) ;
#83341=EDGE_LOOP ( 'NONE', ( #73562, #5299, #45823, #93064 ) ) ;
#83342=DIRECTION ( 'NONE',  ( 0.000000000000000000, 0.000000000000000000, 1.000000000000000000 ) ) ;
#83343=DIRECTION ( 'NONE',  ( 0.000000000000000000, 1.000000000000000000, 0.000000000000000000 ) ) ;
#83344=CARTESIAN_POINT ( 'NONE',  ( -1.850000000000033396, 2.500000000000000000, -6.148780366869526226 ) ) ;
#83345=CARTESIAN_POINT ( 'NONE',  ( 1.899999999999951283, 2.500000000000000000, -4.083716857408426826 ) ) ;
#83346=AXIS2_PLACEMENT_3D ( 'NONE', #127342, #118148, #37670 ) ;
#83347=CARTESIAN_POINT ( 'NONE',  ( -11.24999999999996447, 12.50000000000000000, -6.495190528383298911 ) ) ;
#83348=EDGE_CURVE ( 'NONE', #117173, #59532, #2769, .T. ) ;
#83349=VECTOR ( 'NONE', #102786, 1000.000000000000000 ) ;
#83350=ORIENTED_EDGE ( 'NONE', *, *, #10561, .F. ) ;
#83351=ORIENTED_EDGE ( 'NONE', *, *, #15092, .F. ) ;
#83352=CARTESIAN_POINT ( 'NONE',  ( -8.750000000000010658, 2.500000000000000000, -7.288010851410849256 ) ) ;
#83353=DIRECTION ( 'NONE',  ( 0.000000000000000000, 0.000000000000000000, -1.000000000000000000 ) ) ;
#83354=CIRCLE ( 'NONE', #87529, 0.06509327318403745899 ) ;
#83355=VECTOR ( 'NONE', #732, 1000.000000000000000 ) ;
#83358=CARTESIAN_POINT ( 'NONE',  ( 9.599999999999917932, 2.500000000000000000, -0.1000000000000022815 ) ) ;
#83359=CARTESIAN_POINT ( 'NONE',  ( 9.549999999999915445, 2.500000000000000000, -2.265063509461101798 ) ) ;
#83360=PLANE ( 'NONE',  #45502 ) ;
#83361=VERTEX_POINT ( 'NONE', #91158 ) ;
#83362=CARTESIAN_POINT ( 'NONE',  ( 1.699999999999951994, 2.500000000000000000, -2.276824562219559311E-15 ) ) ;
#83363=DIRECTION ( 'NONE',  ( -0.000000000000000000, -1.000000000000000000, -0.000000000000000000 ) ) ;
#83364=CARTESIAN_POINT ( 'NONE',  ( 0.6499999999999543920, 12.50000000000000000, 6.148780366869520897 ) ) ;
#83366=ORIENTED_EDGE ( 'NONE', *, *, #101397, .F. ) ;
#83367=VECTOR ( 'NONE', #106946, 1000.000000000000000 ) ;
#83368=AXIS2_PLACEMENT_3D ( 'NONE', #85972, #63789, #125902 ) ;
#83369=CARTESIAN_POINT ( 'NONE',  ( 5.399999999999936406, 2.500000000000000000, -4.922947341949753586 ) ) ;
#83370=AXIS2_PLACEMENT_3D ( 'NONE', #75303, #115198, #65477 ) ;
#83371=ORIENTED_EDGE ( 'NONE', *, *, #126116, .F. ) ;
#83372=CARTESIAN_POINT ( 'NONE',  ( 3.349999999999944578, 12.50000000000000000, -1.407149913249512663 ) ) ;
#83373=EDGE_LOOP ( 'NONE', ( #53311, #62377 ) ) ;
#83374=CARTESIAN_POINT ( 'NONE',  ( 9.999999999999914735, 12.50000000000000000, 0.6928203230275494784 ) ) ;
#83375=CIRCLE ( 'NONE', #116803, 0.06509327318403745899 ) ;
#83376=CARTESIAN_POINT ( 'NONE',  ( -5.400000000000020783, 2.500000000000000000, 0.6928203230275494784 ) ) ;
#83377=CARTESIAN_POINT ( 'NONE',  ( -4.800000000000024691, 2.500000000000000000, 4.676537180435972552 ) ) ;
#83378=ORIENTED_EDGE ( 'NONE', *, *, #86906, .T. ) ;
#83379=EDGE_CURVE ( 'NONE', #1899, #66996, #59717, .T. ) ;
#83380=CARTESIAN_POINT ( 'NONE',  ( -2.100000000000033396, 2.500000000000000000, 0.6928203230275494784 ) ) ;
#83381=AXIS2_PLACEMENT_3D ( 'NONE', #68839, #79328, #80607 ) ;
#83382=CONICAL_SURFACE ( 'NONE', #85519, 0.1000000000000002554, 0.003490658503988666988 ) ;
#83383=DIRECTION ( 'NONE',  ( 0.000000000000000000, 0.000000000000000000, -1.000000000000000000 ) ) ;
#83384=AXIS2_PLACEMENT_3D ( 'NONE', #62650, #24003, #114311 ) ;
#83385=EDGE_CURVE ( 'NONE', #107774, #84934, #22438, .T. ) ;
#83386=ADVANCED_FACE ( 'NONE', ( #102271 ), #78672, .T. ) ;
#83387=VERTEX_POINT ( 'NONE', #110785 ) ;
#83389=AXIS2_PLACEMENT_3D ( 'NONE', #105245, #27310, #77704 ) ;
#83390=ORIENTED_EDGE ( 'NONE', *, *, #2569, .T. ) ;
#83391=ORIENTED_EDGE ( 'NONE', *, *, #91944, .T. ) ;
#83392=FACE_OUTER_BOUND ( 'NONE', #80729, .T. ) ;
#83393=DIRECTION ( 'NONE',  ( -0.000000000000000000, 1.000000000000000000, -0.000000000000000000 ) ) ;
#83394=ADVANCED_FACE ( 'NONE', ( #70875 ), #116199, .T. ) ;
#83395=EDGE_CURVE ( 'NONE', #65903, #25992, #43172, .T. ) ;
#83396=CARTESIAN_POINT ( 'NONE',  ( -7.050000000000016698, 12.50000000000000000, -2.165063509461101710 ) ) ;
#83397=ADVANCED_FACE ( 'NONE', ( #89856 ), #20080, .T. ) ;
#83398=ORIENTED_EDGE ( 'NONE', *, *, #47754, .F. ) ;
#83399=EDGE_CURVE ( 'NONE', #25034, #25981, #10629, .T. ) ;
#83400=CARTESIAN_POINT ( 'NONE',  ( 10.84999999999990905, 12.50000000000000000, -6.430097255199264339 ) ) ;
#83401=CARTESIAN_POINT ( 'NONE',  ( 2.299999999999949640, 2.500000000000000000, -4.676537180435977881 ) ) ;
#83402=ORIENTED_EDGE ( 'NONE', *, *, #94944, .T. ) ;
#83403=CARTESIAN_POINT ( 'NONE',  ( -5.600000000000020073, 12.50000000000000000, 4.611443907251934426 ) ) ;
#83404=CARTESIAN_POINT ( 'NONE',  ( 2.500000000000002220, 2.500000000000000000, -8.999999999999998224 ) ) ;
#83405=CARTESIAN_POINT ( 'NONE',  ( -12.94999999999999218, 12.50000000000000000, -2.165063509461099489 ) ) ;
#83406=CARTESIAN_POINT ( 'NONE',  ( -3.550000000000031797, 2.500000000000000000, -6.048780366869526581 ) ) ;
#83407=CIRCLE ( 'NONE', #16476, 0.1000000000000002554 ) ;
#83408=CARTESIAN_POINT ( 'NONE',  ( 9.149999999999916866, 12.50000000000000000, 5.802370205355744659 ) ) ;
#83409=EDGE_CURVE ( 'NONE', #121198, #4792, #103708, .T. ) ;
#83410=DIRECTION ( 'NONE',  ( 0.000000000000000000, 0.000000000000000000, 1.000000000000000000 ) ) ;
#83411=CARTESIAN_POINT ( 'NONE',  ( -13.94999999999998685, 12.50000000000000000, 1.753560074763288013 ) ) ;
#83412=AXIS2_PLACEMENT_3D ( 'NONE', #10410, #109916, #68686 ) ;
#83413=EDGE_LOOP ( 'NONE', ( #47122, #9387 ) ) ;
#83414=ORIENTED_EDGE ( 'NONE', *, *, #65260, .F. ) ;
#83415=ORIENTED_EDGE ( 'NONE', *, *, #12751, .F. ) ;
#83416=VERTEX_POINT ( 'NONE', #53802 ) ;
#83417=CARTESIAN_POINT ( 'NONE',  ( -11.44999999999999751, 2.500000000000000000, 6.148780366869520897 ) ) ;
#83419=DIRECTION ( 'NONE',  ( -4.274815082592931898E-19, -0.9999939076577903929, -0.003490651415223739937 ) ) ;
#83420=ORIENTED_EDGE ( 'NONE', *, *, #23427, .T. ) ;
#83421=FACE_BOUND ( 'NONE', #31270, .T. ) ;
#83422=PLANE ( 'NONE',  #79301 ) ;
#83423=DIRECTION ( 'NONE',  ( 0.000000000000000000, 0.000000000000000000, 1.000000000000000000 ) ) ;
#83424=CIRCLE ( 'NONE', #104340, 0.06509327318403745899 ) ;
#83425=AXIS2_PLACEMENT_3D ( 'NONE', #120971, #129535, #111808 ) ;
#83426=DIRECTION ( 'NONE',  ( 0.000000000000000000, 0.000000000000000000, -1.000000000000000000 ) ) ;
#83427=AXIS2_PLACEMENT_3D ( 'NONE', #107765, #119510, #99251 ) ;
#83428=DIRECTION ( 'NONE',  ( -0.000000000000000000, 1.000000000000000000, -0.000000000000000000 ) ) ;
#83429=CARTESIAN_POINT ( 'NONE',  ( 4.999999999999933387, 2.500000000000000000, 5.022947341949748790 ) ) ;
#83430=DIRECTION ( 'NONE',  ( 0.000000000000000000, 0.000000000000000000, -1.000000000000000000 ) ) ;
#83431=CARTESIAN_POINT ( 'NONE',  ( -13.09999999999999254, 2.500000000000000000, 0.3464101615137777923 ) ) ;
#83432=DIRECTION ( 'NONE',  ( 0.000000000000000000, 0.000000000000000000, 1.000000000000000000 ) ) ;
#83433=EDGE_CURVE ( 'NONE', #128176, #27524, #99595, .T. ) ;
#83434=CARTESIAN_POINT ( 'NONE',  ( -0.2000000000000399791, 2.500000000000000000, -4.776537180435977525 ) ) ;
#83435=AXIS2_PLACEMENT_3D ( 'NONE', #24464, #64380, #87870 ) ;
#83436=DIRECTION ( 'NONE',  ( -4.274815082592931898E-19, -0.9999939076577903929, -0.003490651415223739937 ) ) ;
#83437=ORIENTED_EDGE ( 'NONE', *, *, #69040, .F. ) ;
#83438=AXIS2_PLACEMENT_3D ( 'NONE', #101370, #70612, #3169 ) ;
#83439=VERTEX_POINT ( 'NONE', #115948 ) ;
#83441=ORIENTED_EDGE ( 'NONE', *, *, #15100, .T. ) ;
#83442=ORIENTED_EDGE ( 'NONE', *, *, #76359, .F. ) ;
#83443=ORIENTED_EDGE ( 'NONE', *, *, #17581, .F. ) ;
#83444=EDGE_CURVE ( 'NONE', #61373, #41506, #84914, .T. ) ;
#83445=CARTESIAN_POINT ( 'NONE',  ( -6.050000000000018474, 2.500000000000000000, 6.941600689897073018 ) ) ;
#83446=EDGE_CURVE ( 'NONE', #29292, #10886, #3347, .T. ) ;
#83447=EDGE_LOOP ( 'NONE', ( #38035, #4248, #101284, #70555 ) ) ;
#83448=ORIENTED_EDGE ( 'NONE', *, *, #109740, .T. ) ;
#83449=EDGE_CURVE ( 'NONE', #93629, #5464, #74455, .T. ) ;
#83450=AXIS2_PLACEMENT_3D ( 'NONE', #1481, #182, #51260 ) ;
#83451=EDGE_CURVE ( 'NONE', #42996, #49853, #32711, .T. ) ;
#83452=CARTESIAN_POINT ( 'NONE',  ( 11.44999999999990514, 2.500000000000000000, -6.148780366869526226 ) ) ;
#83453=CARTESIAN_POINT ( 'NONE',  ( -9.150000000000011013, 2.500000000000000000, -5.802370205355744659 ) ) ;
#83454=DIRECTION ( 'NONE',  ( 0.000000000000000000, 0.000000000000000000, 1.000000000000000000 ) ) ;
#83455=CONICAL_SURFACE ( 'NONE', #60479, 0.1000000000000002554, 0.003490658503988666988 ) ;
#83456=EDGE_CURVE ( 'NONE', #20308, #30524, #66124, .T. ) ;
#83457=EDGE_CURVE ( 'NONE', #40017, #13533, #47273, .T. ) ;
#83458=EDGE_LOOP ( 'NONE', ( #105984, #15466, #52080, #87996 ) ) ;
#83459=CARTESIAN_POINT ( 'NONE',  ( 11.69999999999990514, 12.50000000000000000, -2.276824562219559311E-15 ) ) ;
#83460=ADVANCED_FACE ( 'NONE', ( #83899 ), #93242, .T. ) ;
#83461=EDGE_CURVE ( 'NONE', #64597, #68062, #26433, .T. ) ;
#83462=ORIENTED_EDGE ( 'NONE', *, *, #86730, .F. ) ;
#83463=EDGE_CURVE ( 'NONE', #16935, #33066, #84558, .T. ) ;
#83464=ORIENTED_EDGE ( 'NONE', *, *, #76093, .T. ) ;
#83465=CARTESIAN_POINT ( 'NONE',  ( -3.150000000000032330, 2.500000000000000000, -6.148780366869526226 ) ) ;
#83466=FACE_OUTER_BOUND ( 'NONE', #6260, .T. ) ;
#83467=EDGE_LOOP ( 'NONE', ( #55893, #61383 ) ) ;
#83468=AXIS2_PLACEMENT_3D ( 'NONE', #127106, #55134, #45326 ) ;
#83469=ADVANCED_FACE ( 'NONE', ( #23709 ), #1286, .T. ) ;
#83470=ORIENTED_EDGE ( 'NONE', *, *, #34939, .T. ) ;
#83471=CARTESIAN_POINT ( 'NONE',  ( 12.89999999999990266, 12.50000000000000000, -4.957854068765716882 ) ) ;
#83472=AXIS2_PLACEMENT_3D ( 'NONE', #107009, #25897, #76285 ) ;
#83473=DIRECTION ( 'NONE',  ( 0.000000000000000000, 0.000000000000000000, -1.000000000000000000 ) ) ;
#83474=LINE ( 'NONE', #23903, #102237 ) ;
#83475=DIRECTION ( 'NONE',  ( 0.000000000000000000, 1.000000000000000000, 0.000000000000000000 ) ) ;
#83476=CARTESIAN_POINT ( 'NONE',  ( 3.149999999999942624, 12.50000000000000000, 6.148780366869520897 ) ) ;
#83477=VECTOR ( 'NONE', #17242, 1000.000000000000000 ) ;
#83478=ORIENTED_EDGE ( 'NONE', *, *, #17635, .T. ) ;
#83479=DIRECTION ( 'NONE',  ( 0.000000000000000000, 1.000000000000000000, 0.000000000000000000 ) ) ;
#83482=AXIS2_PLACEMENT_3D ( 'NONE', #79053, #50234, #20760 ) ;
#83483=VERTEX_POINT ( 'NONE', #114025 ) ;
#83484=CARTESIAN_POINT ( 'NONE',  ( -1.650000000000034772, 2.500000000000000000, 2.065063509461097624 ) ) ;
#83485=DIRECTION ( 'NONE',  ( 0.000000000000000000, 1.000000000000000000, 0.000000000000000000 ) ) ;
#83486=VECTOR ( 'NONE', #77595, 1000.000000000000000 ) ;
#83487=CARTESIAN_POINT ( 'NONE',  ( -9.600000000000008527, 2.500000000000000000, -3.737306695894645259 ) ) ;
#83488=DIRECTION ( 'NONE',  ( 0.000000000000000000, -0.9999939076577903929, 0.003490651415223739937 ) ) ;
#83489=ORIENTED_EDGE ( 'NONE', *, *, #112991, .F. ) ;
#83490=SURFACE_STYLE_USAGE ( .BOTH. , #94571 ) ;
#83492=CIRCLE ( 'NONE', #35364, 0.1000000000000002554 ) ;
#83493=DIRECTION ( 'NONE',  ( -0.000000000000000000, -1.000000000000000000, -0.000000000000000000 ) ) ;
#83494=ORIENTED_EDGE ( 'NONE', *, *, #126956, .T. ) ;
#83495=EDGE_LOOP ( 'NONE', ( #74381, #17227, #67207, #45628 ) ) ;
#83496=EDGE_LOOP ( 'NONE', ( #97660, #87152 ) ) ;
#83497=PLANE ( 'NONE',  #102229 ) ;
#83498=DIRECTION ( 'NONE',  ( -0.000000000000000000, 1.000000000000000000, -0.000000000000000000 ) ) ;
#83500=CARTESIAN_POINT ( 'NONE',  ( -0.8000000000000381251, 2.500000000000000000, 4.330127018922196314 ) ) ;
#83501=CARTESIAN_POINT ( 'NONE',  ( -8.100000000000013856, 2.500000000000000000, -4.776537180435977525 ) ) ;
#83502=CARTESIAN_POINT ( 'NONE',  ( 87.50000000000001421, 0.000000000000000000, 0.000000000000000000 ) ) ;
#83503=EDGE_CURVE ( 'NONE', #55444, #121877, #5477, .T. ) ;
#83504=FACE_OUTER_BOUND ( 'NONE', #108521, .T. ) ;
#83505=AXIS2_PLACEMENT_3D ( 'NONE', #127843, #77454, #129165 ) ;
#83506=VERTEX_POINT ( 'NONE', #24990 ) ;
#83507=CARTESIAN_POINT ( 'NONE',  ( 9.999999999999911182, 2.500000000000000000, -3.737306695894649700 ) ) ;
#83508=AXIS2_PLACEMENT_3D ( 'NONE', #42471, #110544, #51002 ) ;
#83509=VECTOR ( 'NONE', #41171, 1000.000000000000000 ) ;
#83510=ORIENTED_EDGE ( 'NONE', *, *, #96076, .T. ) ;
#83511=DIRECTION ( 'NONE',  ( 0.000000000000000000, 1.000000000000000000, 0.000000000000000000 ) ) ;
#83512=EDGE_CURVE ( 'NONE', #117253, #92392, #120425, .T. ) ;
#83513=FACE_OUTER_BOUND ( 'NONE', #45360, .T. ) ;
#83515=DIRECTION ( 'NONE',  ( 0.000000000000000000, 0.000000000000000000, -1.000000000000000000 ) ) ;
#83516=ORIENTED_EDGE ( 'NONE', *, *, #53579, .F. ) ;
#83517=AXIS2_PLACEMENT_3D ( 'NONE', #14850, #125478, #33872 ) ;
#83518=AXIS2_PLACEMENT_3D ( 'NONE', #114664, #66205, #74754 ) ;
#83519=LINE ( 'NONE', #104432, #82709 ) ;
#83520=DIRECTION ( 'NONE',  ( -0.000000000000000000, 1.000000000000000000, -0.000000000000000000 ) ) ;
#83521=VERTEX_POINT ( 'NONE', #103565 ) ;
#83522=CONICAL_SURFACE ( 'NONE', #87702, 0.1000000000000000472, 0.003490658503988666988 ) ;
#83523=VERTEX_POINT ( 'NONE', #123204 ) ;
#83524=PLANE ( 'NONE',  #76111 ) ;
#83525=AXIS2_PLACEMENT_3D ( 'NONE', #43440, #42131, #82039 ) ;
#83526=VERTEX_POINT ( 'NONE', #63638 ) ;
#83527=ORIENTED_EDGE ( 'NONE', *, *, #123710, .F. ) ;
#83528=FACE_OUTER_BOUND ( 'NONE', #93648, .T. ) ;
#83529=VERTEX_POINT ( 'NONE', #24355 ) ;
#83530=CARTESIAN_POINT ( 'NONE',  ( 15.44463772192102446, 2.469073678227471813, -4.264595835262737111 ) ) ;
#83531=CARTESIAN_POINT ( 'NONE',  ( -9.150000000000009237, 2.500000000000000000, -1.472243186433550122 ) ) ;
#83532=CARTESIAN_POINT ( 'NONE',  ( -6.450000000000016165, 2.500000000000000000, 2.511473670974873507 ) ) ;
#83533=ORIENTED_EDGE ( 'NONE', *, *, #77912, .F. ) ;
#83534=EDGE_CURVE ( 'NONE', #118050, #16181, #63988, .T. ) ;
#83535=LINE ( 'NONE', #33151, #127780 ) ;
#83537=ORIENTED_EDGE ( 'NONE', *, *, #27847, .T. ) ;
#83538=AXIS2_PLACEMENT_3D ( 'NONE', #111435, #83911, #72824 ) ;
#83539=DIRECTION ( 'NONE',  ( 0.000000000000000000, 0.000000000000000000, 1.000000000000000000 ) ) ;
#83541=ADVANCED_FACE ( 'NONE', ( #64902 ), #104817, .T. ) ;
#83542=ORIENTED_EDGE ( 'NONE', *, *, #54143, .F. ) ;
#83543=ORIENTED_EDGE ( 'NONE', *, *, #27421, .T. ) ;
#83544=ORIENTED_EDGE ( 'NONE', *, *, #46143, .F. ) ;
#83545=EDGE_LOOP ( 'NONE', ( #22060, #74276, #57730, #118369 ) ) ;
#83546=FACE_OUTER_BOUND ( 'NONE', #61325, .T. ) ;
#83547=CARTESIAN_POINT ( 'NONE',  ( 3.709550432166843770, 1.500000000000382583, 10.00000000000000533 ) ) ;
#83548=EDGE_CURVE ( 'NONE', #84561, #121566, #36810, .T. ) ;
#83549=ADVANCED_FACE ( 'NONE', ( #75366 ), #68177, .T. ) ;
#83550=FACE_OUTER_BOUND ( 'NONE', #6414, .T. ) ;
#83552=FACE_BOUND ( 'NONE', #48981, .T. ) ;
#83553=EDGE_LOOP ( 'NONE', ( #20085, #34280 ) ) ;
#83554=EDGE_CURVE ( 'NONE', #4826, #5152, #39351, .T. ) ;
#83556=EDGE_CURVE ( 'NONE', #31381, #19741, #76675, .T. ) ;
#83557=DIRECTION ( 'NONE',  ( 0.000000000000000000, 0.000000000000000000, -1.000000000000000000 ) ) ;
#83558=DIRECTION ( 'NONE',  ( 0.000000000000000000, -0.9999939076577903929, 0.003490651415223739937 ) ) ;
#83559=LINE ( 'NONE', #43011, #4642 ) ;
#83561=CIRCLE ( 'NONE', #125407, 0.06509327318403745899 ) ;
#83562=EDGE_CURVE ( 'NONE', #73190, #7558, #97426, .T. ) ;
#83563=DIRECTION ( 'NONE',  ( -0.000000000000000000, -1.000000000000000000, -0.000000000000000000 ) ) ;
#83564=EDGE_CURVE ( 'NONE', #80681, #55060, #61941, .T. ) ;
#83565=ADVANCED_FACE ( 'NONE', ( #7915 ), #41025, .T. ) ;
#83566=FACE_OUTER_BOUND ( 'NONE', #68955, .T. ) ;
#83567=CIRCLE ( 'NONE', #39758, 0.06509327318403745899 ) ;
#83568=AXIS2_PLACEMENT_3D ( 'NONE', #55376, #86756, #27836 ) ;
#83569=ORIENTED_EDGE ( 'NONE', *, *, #52943, .T. ) ;
#83570=ORIENTED_EDGE ( 'NONE', *, *, #51336, .T. ) ;
#83571=ORIENTED_EDGE ( 'NONE', *, *, #10980, .F. ) ;
#83572=ORIENTED_EDGE ( 'NONE', *, *, #99262, .F. ) ;
#83573=EDGE_LOOP ( 'NONE', ( #33625, #118602 ) ) ;
#83574=DIRECTION ( 'NONE',  ( 0.000000000000000000, 0.000000000000000000, 1.000000000000000000 ) ) ;
#83575=CIRCLE ( 'NONE', #27132, 0.09999999999999982514 ) ;
#83576=FACE_OUTER_BOUND ( 'NONE', #126265, .T. ) ;
#83577=ORIENTED_EDGE ( 'NONE', *, *, #8457, .F. ) ;
#83578=FACE_BOUND ( 'NONE', #70260, .T. ) ;
#83579=LINE ( 'NONE', #54732, #123091 ) ;
#83580=CONICAL_SURFACE ( 'NONE', #4125, 0.1000000000000002554, 0.003490658503988666988 ) ;
#83581=CIRCLE ( 'NONE', #27138, 0.09999999999999982514 ) ;
#83582=ORIENTED_EDGE ( 'NONE', *, *, #58484, .F. ) ;
#83583=DIRECTION ( 'NONE',  ( -1.000000000000000000, -0.000000000000000000, -0.000000000000000000 ) ) ;
#83584=LINE ( 'NONE', #123482, #99181 ) ;
#83585=DIRECTION ( 'NONE',  ( 0.000000000000000000, 1.000000000000000000, 0.000000000000000000 ) ) ;
#83586=ORIENTED_EDGE ( 'NONE', *, *, #109698, .T. ) ;
#83587=DIRECTION ( 'NONE',  ( -0.000000000000000000, -1.000000000000000000, -0.000000000000000000 ) ) ;
#83588=EDGE_LOOP ( 'NONE', ( #43529, #124147 ) ) ;
#83589=ORIENTED_EDGE ( 'NONE', *, *, #85790, .T. ) ;
#83590=ORIENTED_EDGE ( 'NONE', *, *, #109733, .F. ) ;
#83591=DIRECTION ( 'NONE',  ( -4.274815082592931898E-19, -0.9999939076577903929, -0.003490651415223739937 ) ) ;
#83592=CARTESIAN_POINT ( 'NONE',  ( 2.499999999999948930, 2.500000000000000000, -0.6928203230275541413 ) ) ;
#83593=DIRECTION ( 'NONE',  ( 0.000000000000000000, 1.000000000000000000, 0.000000000000000000 ) ) ;
#83594=EDGE_LOOP ( 'NONE', ( #106801, #127472, #39845, #14024 ) ) ;
#83595=DIRECTION ( 'NONE',  ( -0.000000000000000000, -1.000000000000000000, -0.000000000000000000 ) ) ;
#83596=CARTESIAN_POINT ( 'NONE',  ( 12.04999999999990834, 2.500000000000000000, 6.595190528383296780 ) ) ;
#83598=DIRECTION ( 'NONE',  ( 0.000000000000000000, 0.000000000000000000, -1.000000000000000000 ) ) ;
#83600=ORIENTED_EDGE ( 'NONE', *, *, #26484, .F. ) ;
#83601=CARTESIAN_POINT ( 'NONE',  ( 6.849999999999929479, 2.500000000000000000, 6.941600689897073018 ) ) ;
#83602=EDGE_CURVE ( 'NONE', #90022, #12489, #24271, .T. ) ;
#83603=ORIENTED_EDGE ( 'NONE', *, *, #79409, .F. ) ;
#83604=CARTESIAN_POINT ( 'NONE',  ( -6.450000000000016165, 12.50000000000000000, 6.841600689897072485 ) ) ;
#83605=VECTOR ( 'NONE', #90357, 1000.000000000000000 ) ;
#83606=EDGE_CURVE ( 'NONE', #41921, #116415, #79263, .T. ) ;
#83607=ORIENTED_EDGE ( 'NONE', *, *, #22712, .F. ) ;
#83608=ADVANCED_FACE ( 'NONE', ( #8548 ), #120517, .T. ) ;
#83609=ORIENTED_EDGE ( 'NONE', *, *, #90543, .T. ) ;
#83610=DIRECTION ( 'NONE',  ( 0.000000000000000000, -0.000000000000000000, 1.000000000000000000 ) ) ;
#83611=CARTESIAN_POINT ( 'NONE',  ( -8.150000000000009237, 2.500000000000000000, 6.148780366869520009 ) ) ;
#83612=DIRECTION ( 'NONE',  ( -0.000000000000000000, -1.000000000000000000, -0.000000000000000000 ) ) ;
#83613=DIRECTION ( 'NONE',  ( 0.000000000000000000, 1.000000000000000000, 0.000000000000000000 ) ) ;
#83614=FACE_OUTER_BOUND ( 'NONE', #11949, .T. ) ;
#83615=VERTEX_POINT ( 'NONE', #38033 ) ;
#83616=EDGE_CURVE ( 'NONE', #69443, #55889, #18386, .T. ) ;
#83617=ORIENTED_EDGE ( 'NONE', *, *, #100222, .T. ) ;
#83618=CONICAL_SURFACE ( 'NONE', #45967, 0.09999999999999982514, 0.003490658503988666988 ) ;
#83619=DIRECTION ( 'NONE',  ( 0.000000000000000000, -0.9999939076577903929, 0.003490651415223739937 ) ) ;
#83620=VECTOR ( 'NONE', #43303, 1000.000000000000000 ) ;
#83621=CARTESIAN_POINT ( 'NONE',  ( 5.399999999999932854, 2.500000000000000000, 4.922947341949748257 ) ) ;
#83624=ORIENTED_EDGE ( 'NONE', *, *, #122540, .F. ) ;
#83625=VECTOR ( 'NONE', #116578, 1000.000000000000000 ) ;
#83626=DIRECTION ( 'NONE',  ( 0.000000000000000000, 0.000000000000000000, -1.000000000000000000 ) ) ;
#83627=AXIS2_PLACEMENT_3D ( 'NONE', #26036, #5725, #106517 ) ;
#83628=ORIENTED_EDGE ( 'NONE', *, *, #14658, .T. ) ;
#83629=CARTESIAN_POINT ( 'NONE',  ( 5.649999999999934630, 2.500000000000000000, -2.611473670974877592 ) ) ;
#83631=VERTEX_POINT ( 'NONE', #47868 ) ;
#83632=DIRECTION ( 'NONE',  ( -0.000000000000000000, -1.000000000000000000, -0.000000000000000000 ) ) ;
#83633=FACE_OUTER_BOUND ( 'NONE', #52802, .T. ) ;
#83634=VECTOR ( 'NONE', #127654, 1000.000000000000000 ) ;
#83635=PLANE ( 'NONE',  #65582 ) ;
#83637=DIRECTION ( 'NONE',  ( 0.000000000000000000, 0.000000000000000000, -1.000000000000000000 ) ) ;
#83638=ORIENTED_EDGE ( 'NONE', *, *, #128667, .F. ) ;
#83639=CARTESIAN_POINT ( 'NONE',  ( 2.699999999999946443, 12.50000000000000000, 0.3464101615137735735 ) ) ;
#83640=CARTESIAN_POINT ( 'NONE',  ( 10.19999999999991225, 2.500000000000000000, -4.576537180435978236 ) ) ;
#83641=ORIENTED_EDGE ( 'NONE', *, *, #89636, .T. ) ;
#83644=CARTESIAN_POINT ( 'NONE',  ( -6.650000000000014566, 2.500000000000000000, 6.595190528383296780 ) ) ;
#83645=DIRECTION ( 'NONE',  ( -0.000000000000000000, 1.000000000000000000, -0.000000000000000000 ) ) ;
#83646=CARTESIAN_POINT ( 'NONE',  ( 13.74999999999989519, 12.50000000000000000, -2.857883832488653741 ) ) ;
#83647=DIRECTION ( 'NONE',  ( 0.000000000000000000, -0.9999939076577903929, 0.003490651415223739937 ) ) ;
#83648=CARTESIAN_POINT ( 'NONE',  ( -9.150000000000009237, 2.500000000000000000, -6.395190528383296602 ) ) ;
#83649=CARTESIAN_POINT ( 'NONE',  ( -7.500000000000001776, 1.500000000000000000, 1.734723475976807094E-15 ) ) ;
#83650=EDGE_CURVE ( 'NONE', #68081, #3295, #87761, .T. ) ;
#83651=CARTESIAN_POINT ( 'NONE',  ( -4.400000000000025224, 2.500000000000000000, 3.983716857408420076 ) ) ;
#83652=CARTESIAN_POINT ( 'NONE',  ( -7.499999999999980460, 12.50000000000000000, -2.276824562219559311E-15 ) ) ;
#83653=LINE ( 'NONE', #60321, #115184 ) ;
#83654=CIRCLE ( 'NONE', #75230, 0.06509327318403745899 ) ;
#83655=DIRECTION ( 'NONE',  ( 0.000000000000000000, 0.000000000000000000, 1.000000000000000000 ) ) ;
#83656=ORIENTED_EDGE ( 'NONE', *, *, #7492, .T. ) ;
#83657=ORIENTED_EDGE ( 'NONE', *, *, #75288, .F. ) ;
#83658=AXIS2_PLACEMENT_3D ( 'NONE', #128655, #38990, #118798 ) ;
#83659=EDGE_LOOP ( 'NONE', ( #14982, #91184 ) ) ;
#83661=ADVANCED_FACE ( 'NONE', ( #88404 ), #36763, .T. ) ;
#83662=FACE_OUTER_BOUND ( 'NONE', #83734, .T. ) ;
#83663=LINE ( 'NONE', #127295, #129424 ) ;
#83664=CIRCLE ( 'NONE', #14590, 0.06509327318403745899 ) ;
#83665=ORIENTED_EDGE ( 'NONE', *, *, #3150, .T. ) ;
#83666=DIRECTION ( 'NONE',  ( 0.000000000000000000, 1.000000000000000000, 0.000000000000000000 ) ) ;
#83667=DIRECTION ( 'NONE',  ( 0.000000000000000000, 0.000000000000000000, 1.000000000000000000 ) ) ;
#83668=CARTESIAN_POINT ( 'NONE',  ( -11.84999999999999609, 12.50000000000000000, 1.818653347947321475 ) ) ;
#83669=ORIENTED_EDGE ( 'NONE', *, *, #322, .T. ) ;
#83670=DIRECTION ( 'NONE',  ( 0.000000000000000000, 1.000000000000000000, 0.000000000000000000 ) ) ;
#83671=FACE_OUTER_BOUND ( 'NONE', #87933, .T. ) ;
#83672=ORIENTED_EDGE ( 'NONE', *, *, #100227, .T. ) ;
#83673=ORIENTED_EDGE ( 'NONE', *, *, #11145, .F. ) ;
#83674=VERTEX_POINT ( 'NONE', #9218 ) ;
#83675=ORIENTED_EDGE ( 'NONE', *, *, #101872, .T. ) ;
#83676=DIRECTION ( 'NONE',  ( -0.000000000000000000, 1.000000000000000000, -0.000000000000000000 ) ) ;
#83677=CARTESIAN_POINT ( 'NONE',  ( -15.19999999999998153, 2.500000000000000000, -0.3464101615137759604 ) ) ;
#83678=CARTESIAN_POINT ( 'NONE',  ( 4.199999999999941558, 2.500000000000000000, -4.330127018922201643 ) ) ;
#83679=DIRECTION ( 'NONE',  ( 0.000000000000000000, 0.000000000000000000, 1.000000000000000000 ) ) ;
#83680=CIRCLE ( 'NONE', #14695, 0.06509327318403743123 ) ;
#83681=ORIENTED_EDGE ( 'NONE', *, *, #96396, .T. ) ;
#83682=AXIS2_PLACEMENT_3D ( 'NONE', #59127, #119312, #47367 ) ;
#83683=EDGE_CURVE ( 'NONE', #41491, #118121, #28871, .T. ) ;
#83684=DIRECTION ( 'NONE',  ( 0.000000000000000000, -0.9999939076577903929, 0.003490651415223739937 ) ) ;
#83685=VERTEX_POINT ( 'NONE', #108703 ) ;
#83686=DIRECTION ( 'NONE',  ( 0.000000000000000000, 0.000000000000000000, 1.000000000000000000 ) ) ;
#83688=CARTESIAN_POINT ( 'NONE',  ( -6.050000000000020250, 2.500000000000000000, -6.741600689897078169 ) ) ;
#83689=DIRECTION ( 'NONE',  ( 0.000000000000000000, -0.9999939076577903929, 0.003490651415223739937 ) ) ;
#83690=ADVANCED_FACE ( 'NONE', ( #19019 ), #49166, .T. ) ;
#83692=EDGE_CURVE ( 'NONE', #106597, #18843, #27545, .T. ) ;
#83693=ORIENTED_EDGE ( 'NONE', *, *, #126096, .T. ) ;
#83694=EDGE_LOOP ( 'NONE', ( #28894, #104447, #33503, #87723 ) ) ;
#83695=ORIENTED_EDGE ( 'NONE', *, *, #38304, .F. ) ;
#83696=DIRECTION ( 'NONE',  ( -0.000000000000000000, -1.000000000000000000, -0.000000000000000000 ) ) ;
#83697=DIRECTION ( 'NONE',  ( 0.000000000000000000, -0.9999939076577903929, 0.003490651415223739937 ) ) ;
#83698=ADVANCED_FACE ( 'NONE', ( #26928 ), #67462, .T. ) ;
#83699=EDGE_CURVE ( 'NONE', #122964, #43427, #43263, .T. ) ;
#83700=DIRECTION ( 'NONE',  ( 0.000000000000000000, 0.000000000000000000, 1.000000000000000000 ) ) ;
#83701=ADVANCED_FACE ( 'NONE', ( #111933 ), #82960, .T. ) ;
#83702=FACE_BOUND ( 'NONE', #103015, .T. ) ;
#83703=ADVANCED_FACE ( 'NONE', ( #41913 ), #52363, .T. ) ;
#83704=DIRECTION ( 'NONE',  ( 0.000000000000000000, 1.000000000000000000, 0.000000000000000000 ) ) ;
#83705=CARTESIAN_POINT ( 'NONE',  ( -8.950000000000006395, 2.500000000000000000, 6.741600689897071952 ) ) ;
#83706=DIRECTION ( 'NONE',  ( -0.000000000000000000, 1.000000000000000000, -0.000000000000000000 ) ) ;
#83707=AXIS2_PLACEMENT_3D ( 'NONE', #59043, #30244, #110701 ) ;
#83708=AXIS2_PLACEMENT_3D ( 'NONE', #86904, #7693, #109779 ) ;
#83709=EDGE_CURVE ( 'NONE', #110285, #24530, #124715, .T. ) ;
#83710=CARTESIAN_POINT ( 'NONE',  ( 1.049999999999953637, 2.500000000000000000, -1.818653347947326138 ) ) ;
#83711=EDGE_CURVE ( 'NONE', #52810, #8036, #93328, .T. ) ;
#83712=DIRECTION ( 'NONE',  ( 0.000000000000000000, 1.000000000000000000, 0.000000000000000000 ) ) ;
#83713=EDGE_CURVE ( 'NONE', #85857, #53445, #87049, .T. ) ;
#83714=CARTESIAN_POINT ( 'NONE',  ( 0.3999999999999628852, 2.500000000000000000, 0.7928203230275517877 ) ) ;
#83715=VERTEX_POINT ( 'NONE', #102112 ) ;
#83716=CIRCLE ( 'NONE', #39813, 0.1000000000000002554 ) ;
#83717=ADVANCED_FACE ( 'NONE', ( #100181 ), #57826, .T. ) ;
#83718=EDGE_CURVE ( 'NONE', #58034, #110840, #114248, .T. ) ;
#83719=CARTESIAN_POINT ( 'NONE',  ( -2.100000000000034728, 2.500000000000000000, 4.330127018922196314 ) ) ;
#83720=VERTEX_POINT ( 'NONE', #82483 ) ;
#83721=ORIENTED_EDGE ( 'NONE', *, *, #95137, .T. ) ;
#83722=ORIENTED_EDGE ( 'NONE', *, *, #3445, .F. ) ;
#83723=ORIENTED_EDGE ( 'NONE', *, *, #80873, .F. ) ;
#83724=PLANE ( 'NONE',  #8932 ) ;
#83725=FACE_BOUND ( 'NONE', #31489, .T. ) ;
#83726=EDGE_CURVE ( 'NONE', #104677, #62516, #41114, .T. ) ;
#83727=DIRECTION ( 'NONE',  ( -0.000000000000000000, 1.000000000000000000, -0.000000000000000000 ) ) ;
#83728=ORIENTED_EDGE ( 'NONE', *, *, #115750, .F. ) ;
#83729=CARTESIAN_POINT ( 'NONE',  ( -11.44999999999999751, 2.500000000000000000, 2.411473670974873862 ) ) ;
#83732=LINE ( 'NONE', #95477, #40683 ) ;
#83733=FACE_OUTER_BOUND ( 'NONE', #119985, .T. ) ;
#83734=EDGE_LOOP ( 'NONE', ( #12411, #39307, #10530, #117329 ) ) ;
#83735=LINE ( 'NONE', #85660, #36058 ) ;
#83736=CONICAL_SURFACE ( 'NONE', #27289, 0.1000000000000000472, 0.003490658503988666988 ) ;
#83737=FACE_OUTER_BOUND ( 'NONE', #55367, .T. ) ;
#83738=EDGE_LOOP ( 'NONE', ( #13036, #78649 ) ) ;
#83739=DIRECTION ( 'NONE',  ( 0.000000000000000000, 0.000000000000000000, -1.000000000000000000 ) ) ;
#83740=CONICAL_SURFACE ( 'NONE', #2242, 0.1000000000000002554, 0.003490658503988666988 ) ;
#83741=CARTESIAN_POINT ( 'NONE',  ( 4.349999999999940137, 2.500000000000000000, -2.411473670974877859 ) ) ;
#83742=DIRECTION ( 'NONE',  ( 0.000000000000000000, 1.000000000000000000, 0.000000000000000000 ) ) ;
#83743=ORIENTED_EDGE ( 'NONE', *, *, #20603, .T. ) ;
#83744=ORIENTED_EDGE ( 'NONE', *, *, #28582, .T. ) ;
#83745=DIRECTION ( 'NONE',  ( 0.000000000000000000, -0.000000000000000000, 1.000000000000000000 ) ) ;
#83746=ORIENTED_EDGE ( 'NONE', *, *, #46811, .T. ) ;
#83747=FACE_OUTER_BOUND ( 'NONE', #122836, .T. ) ;
#83748=CARTESIAN_POINT ( 'NONE',  ( 0.1999999999999636513, 12.50000000000000000, -0.3464101615137760715 ) ) ;
#83749=EDGE_CURVE ( 'NONE', #38510, #24704, #118447, .T. ) ;
#83750=ORIENTED_EDGE ( 'NONE', *, *, #40412, .T. ) ;
#83751=FACE_OUTER_BOUND ( 'NONE', #6316, .T. ) ;
#83752=EDGE_CURVE ( 'NONE', #90411, #63793, #74542, .T. ) ;
#83753=DIRECTION ( 'NONE',  ( 0.000000000000000000, 0.000000000000000000, -1.000000000000000000 ) ) ;
#83754=FACE_OUTER_BOUND ( 'NONE', #1944, .T. ) ;
#83755=DIRECTION ( 'NONE',  ( -0.000000000000000000, 1.000000000000000000, -0.000000000000000000 ) ) ;
#83756=CARTESIAN_POINT ( 'NONE',  ( 1.649999999999951505, 2.500000000000000000, 1.372243186433545370 ) ) ;
#83757=ADVANCED_FACE ( 'NONE', ( #49805 ), #47360, .T. ) ;
#83758=ORIENTED_EDGE ( 'NONE', *, *, #78213, .F. ) ;
#83759=EDGE_LOOP ( 'NONE', ( #72864, #109227 ) ) ;
#83760=CARTESIAN_POINT ( 'NONE',  ( 1.249999999999950262, 2.500000000000000000, 7.188010851410848723 ) ) ;
#83761=CARTESIAN_POINT ( 'NONE',  ( 9.999999999999912959, 12.50000000000000000, -5.022947341949754119 ) ) ;
#83762=ORIENTED_EDGE ( 'NONE', *, *, #20561, .F. ) ;
#83763=EDGE_LOOP ( 'NONE', ( #112478, #86797, #128713, #20845 ) ) ;
#83764=EDGE_LOOP ( 'NONE', ( #12522, #108016 ) ) ;
#83765=CARTESIAN_POINT ( 'NONE',  ( 7.899999999999924860, 2.500000000000000000, -4.330127018922201643 ) ) ;
#83771=DIRECTION ( 'NONE',  ( 0.000000000000000000, 0.000000000000000000, -1.000000000000000000 ) ) ;
#83772=DIRECTION ( 'NONE',  ( -0.000000000000000000, -1.000000000000000000, -0.000000000000000000 ) ) ;
#83773=FACE_OUTER_BOUND ( 'NONE', #19027, .T. ) ;
#83774=CARTESIAN_POINT ( 'NONE',  ( 6.849999999999929479, 2.500000000000000000, 6.048780366869520364 ) ) ;
#83775=CARTESIAN_POINT ( 'NONE',  ( -11.89999999999999680, 2.500000000000000000, -0.4464101615137742174 ) ) ;
#83776=DIRECTION ( 'NONE',  ( 0.000000000000000000, 1.000000000000000000, 0.000000000000000000 ) ) ;
#83777=ORIENTED_EDGE ( 'NONE', *, *, #59324, .F. ) ;
#83778=DIRECTION ( 'NONE',  ( 0.000000000000000000, 0.000000000000000000, 1.000000000000000000 ) ) ;
#83779=VERTEX_POINT ( 'NONE', #39976 ) ;
#83780=EDGE_LOOP ( 'NONE', ( #80071, #64984, #66430, #19495 ) ) ;
#83781=DIRECTION ( 'NONE',  ( 0.000000000000000000, 0.000000000000000000, 1.000000000000000000 ) ) ;
#83782=FACE_OUTER_BOUND ( 'NONE', #27859, .T. ) ;
#83783=PLANE ( 'NONE',  #100904 ) ;
#83784=CIRCLE ( 'NONE', #117206, 0.1000000000000002554 ) ;
#83785=EDGE_CURVE ( 'NONE', #127462, #82307, #84995, .T. ) ;
#83786=DIRECTION ( 'NONE',  ( -0.000000000000000000, 1.000000000000000000, -0.000000000000000000 ) ) ;
#83787=AXIS2_PLACEMENT_3D ( 'NONE', #125396, #25906, #63898 ) ;
#83788=DIRECTION ( 'NONE',  ( -0.000000000000000000, -1.000000000000000000, -0.000000000000000000 ) ) ;
#83789=CARTESIAN_POINT ( 'NONE',  ( 10.39999999999991154, 12.50000000000000000, -5.088040615133791356 ) ) ;
#83790=DIRECTION ( 'NONE',  ( 0.000000000000000000, 0.000000000000000000, 1.000000000000000000 ) ) ;
#83791=EDGE_LOOP ( 'NONE', ( #78372, #52406, #85651, #39864 ) ) ;
#83792=CARTESIAN_POINT ( 'NONE',  ( -8.750000000000008882, 2.500000000000000000, 1.472243186433545459 ) ) ;
#83793=DIRECTION ( 'NONE',  ( 0.000000000000000000, -0.9999939076577903929, 0.003490651415223739937 ) ) ;
#83794=VERTEX_POINT ( 'NONE', #79888 ) ;
#83795=ORIENTED_EDGE ( 'NONE', *, *, #86145, .F. ) ;
#83796=AXIS2_PLACEMENT_3D ( 'NONE', #36243, #14631, #65681 ) ;
#83797=EDGE_LOOP ( 'NONE', ( #20848, #75148, #84625, #75153 ) ) ;
#83798=ADVANCED_FACE ( 'NONE', ( #20968 ), #71341, .T. ) ;
#83799=EDGE_CURVE ( 'NONE', #96482, #124893, #64079, .T. ) ;
#83800=VERTEX_POINT ( 'NONE', #80547 ) ;
#83801=DIRECTION ( 'NONE',  ( 0.000000000000000000, 1.000000000000000000, 0.000000000000000000 ) ) ;
#83802=CARTESIAN_POINT ( 'NONE',  ( 9.799999999999918998, 12.50000000000000000, -0.3464101615137782364 ) ) ;
#83803=CARTESIAN_POINT ( 'NONE',  ( -15.39999999999998082, 2.500000000000000000, 0.6928203230275518099 ) ) ;
#83804=DIRECTION ( 'NONE',  ( 0.000000000000000000, 0.000000000000000000, -1.000000000000000000 ) ) ;
#83805=LINE ( 'NONE', #54991, #34607 ) ;
#83806=EDGE_LOOP ( 'NONE', ( #43778, #102982, #59186, #126784 ) ) ;
#83807=CARTESIAN_POINT ( 'NONE',  ( -13.54999999999999005, 2.500000000000000000, -1.818653347947323917 ) ) ;
#83808=EDGE_CURVE ( 'NONE', #72985, #37773, #7630, .T. ) ;
#83809=DIRECTION ( 'NONE',  ( 0.000000000000000000, 0.000000000000000000, 1.000000000000000000 ) ) ;
#83810=CARTESIAN_POINT ( 'NONE',  ( -3.150000000000030553, 2.500000000000000000, 6.248780366869520542 ) ) ;
#83811=CARTESIAN_POINT ( 'NONE',  ( -8.749999999999976907, 12.50000000000000000, -6.495190528383297135 ) ) ;
#83812=ORIENTED_EDGE ( 'NONE', *, *, #94784, .T. ) ;
#83813=ORIENTED_EDGE ( 'NONE', *, *, #94601, .T. ) ;
#83814=VERTEX_POINT ( 'NONE', #101470 ) ;
#83815=CIRCLE ( 'NONE', #125570, 0.06509327318403745899 ) ;
#83817=CONICAL_SURFACE ( 'NONE', #85864, 0.1000000000000000056, 0.003490658503988666988 ) ;
#83818=FACE_OUTER_BOUND ( 'NONE', #45301, .T. ) ;
#83819=DIRECTION ( 'NONE',  ( -0.000000000000000000, -1.000000000000000000, -0.000000000000000000 ) ) ;
#83820=AXIS2_PLACEMENT_3D ( 'NONE', #125043, #15723, #35385 ) ;
#83821=EDGE_LOOP ( 'NONE', ( #54976, #89590 ) ) ;
#83822=CARTESIAN_POINT ( 'NONE',  ( 10.39999999999990976, 12.50000000000000000, 4.395220292106234439 ) ) ;
#83823=CARTESIAN_POINT ( 'NONE',  ( 12.94999999999989981, 2.500000000000000000, -2.165063509461101710 ) ) ;
#83824=DIRECTION ( 'NONE',  ( 0.000000000000000000, 1.000000000000000000, 0.000000000000000000 ) ) ;
#83825=DIRECTION ( 'NONE',  ( 0.000000000000000000, -0.9999939076577903929, 0.003490651415223739937 ) ) ;
#83826=EDGE_CURVE ( 'NONE', #49661, #61872, #60890, .T. ) ;
#83827=DIRECTION ( 'NONE',  ( 0.000000000000000000, 1.000000000000000000, 0.000000000000000000 ) ) ;
#83828=ORIENTED_EDGE ( 'NONE', *, *, #30551, .T. ) ;
#83829=ORIENTED_EDGE ( 'NONE', *, *, #103952, .T. ) ;
#83830=ADVANCED_FACE ( 'NONE', ( #124331 ), #64752, .T. ) ;
#83831=CARTESIAN_POINT ( 'NONE',  ( 15.83209681635555022, -2.500000000000000000, -5.404881881984138658 ) ) ;
#83832=CARTESIAN_POINT ( 'NONE',  ( -6.450000000000016165, 2.500000000000000000, 2.511473670974873507 ) ) ;
#83833=EDGE_CURVE ( 'NONE', #73941, #61976, #54929, .T. ) ;
#83834=CARTESIAN_POINT ( 'NONE',  ( -4.150000000000027889, 2.500000000000000000, -7.188010851410854052 ) ) ;
#83837=EDGE_LOOP ( 'NONE', ( #94717, #21298 ) ) ;
#83839=EDGE_CURVE ( 'NONE', #36746, #126920, #93581, .T. ) ;
#83840=ORIENTED_EDGE ( 'NONE', *, *, #64835, .T. ) ;
#83841=FACE_OUTER_BOUND ( 'NONE', #106436, .T. ) ;
#83842=DIRECTION ( 'NONE',  ( 0.000000000000000000, -0.000000000000000000, 1.000000000000000000 ) ) ;
#83843=EDGE_CURVE ( 'NONE', #107104, #52720, #13053, .T. ) ;
#83844=DIRECTION ( 'NONE',  ( 0.000000000000000000, -0.000000000000000000, 1.000000000000000000 ) ) ;
#83845=CARTESIAN_POINT ( 'NONE',  ( 4.149999999999939959, 12.50000000000000000, 2.792790559304612064 ) ) ;
#83846=ORIENTED_EDGE ( 'NONE', *, *, #24456, .T. ) ;
#83847=AXIS2_PLACEMENT_3D ( 'NONE', #4567, #44522, #124386 ) ;
#83848=DIRECTION ( 'NONE',  ( 0.000000000000000000, 1.000000000000000000, 0.000000000000000000 ) ) ;
#83849=AXIS2_PLACEMENT_3D ( 'NONE', #49513, #51449, #90049 ) ;
#83850=EDGE_CURVE ( 'NONE', #40065, #26773, #116386, .T. ) ;
#83851=LINE ( 'NONE', #123147, #114187 ) ;
#83852=ORIENTED_EDGE ( 'NONE', *, *, #115771, .F. ) ;
#83853=CARTESIAN_POINT ( 'NONE',  ( 10.19999999999991047, 2.500000000000000000, 4.576537180435972019 ) ) ;
#83854=VERTEX_POINT ( 'NONE', #103402 ) ;
#83856=EDGE_CURVE ( 'NONE', #55517, #18996, #20162, .T. ) ;
#83857=CARTESIAN_POINT ( 'NONE',  ( -14.14999999999998792, 12.50000000000000000, -1.472243186433547901 ) ) ;
#83858=VECTOR ( 'NONE', #38071, 1000.000000000000000 ) ;
#83859=ORIENTED_EDGE ( 'NONE', *, *, #7505, .T. ) ;
#83860=DIRECTION ( 'NONE',  ( 0.000000000000000000, 1.000000000000000000, 0.000000000000000000 ) ) ;
#83861=CARTESIAN_POINT ( 'NONE',  ( 12.09999999999990195, 2.500000000000000000, -2.276824562219559311E-15 ) ) ;
#83862=ORIENTED_EDGE ( 'NONE', *, *, #107375, .F. ) ;
#83863=ORIENTED_EDGE ( 'NONE', *, *, #110405, .F. ) ;
#83865=PLANE ( 'NONE',  #106267 ) ;
#83866=VECTOR ( 'NONE', #98627, 1000.000000000000000 ) ;
#83869=CIRCLE ( 'NONE', #119377, 0.1000000000000002554 ) ;
#83870=DIRECTION ( 'NONE',  ( 0.000000000000000000, 0.000000000000000000, 1.000000000000000000 ) ) ;
#83871=DIRECTION ( 'NONE',  ( 0.000000000000000000, 0.000000000000000000, 1.000000000000000000 ) ) ;
#83872=PLANE ( 'NONE',  #114295 ) ;
#83873=LINE ( 'NONE', #5311, #84069 ) ;
#83874=VERTEX_POINT ( 'NONE', #104666 ) ;
#83875=VERTEX_POINT ( 'NONE', #14353 ) ;
#83876=CARTESIAN_POINT ( 'NONE',  ( 12.29999999999990301, 2.500000000000000000, -0.3464101615137782364 ) ) ;
#83877=VERTEX_POINT ( 'NONE', #92944 ) ;
#83878=CIRCLE ( 'NONE', #125724, 0.06509327318403745899 ) ;
#83879=AXIS2_PLACEMENT_3D ( 'NONE', #14218, #54170, #37111 ) ;
#83880=DIRECTION ( 'NONE',  ( 0.000000000000000000, 0.000000000000000000, -1.000000000000000000 ) ) ;
#83881=CARTESIAN_POINT ( 'NONE',  ( -8.350000000000013856, 12.50000000000000000, 2.230156782645134950 ) ) ;
#83882=CARTESIAN_POINT ( 'NONE',  ( 4.349999999999938360, 12.50000000000000000, 1.818653347947321475 ) ) ;
#83883=ORIENTED_EDGE ( 'NONE', *, *, #78984, .T. ) ;
#83884=ORIENTED_EDGE ( 'NONE', *, *, #68461, .T. ) ;
#83885=FACE_BOUND ( 'NONE', #19530, .T. ) ;
#83886=VERTEX_POINT ( 'NONE', #3266 ) ;
#83887=CARTESIAN_POINT ( 'NONE',  ( 14.79999999999989413, 12.50000000000000000, -0.3464101615137782364 ) ) ;
#83888=DIRECTION ( 'NONE',  ( -0.000000000000000000, -1.000000000000000000, -0.000000000000000000 ) ) ;
#83890=CARTESIAN_POINT ( 'NONE',  ( 8.349999999999923261, 12.50000000000000000, 1.472243186433545459 ) ) ;
#83891=DIRECTION ( 'NONE',  ( 0.000000000000000000, 1.000000000000000000, 0.000000000000000000 ) ) ;
#83893=CARTESIAN_POINT ( 'NONE',  ( -5.200000000000024158, 2.500000000000000000, -4.676537180435977881 ) ) ;
#83894=DIRECTION ( 'NONE',  ( 0.000000000000000000, 1.000000000000000000, 0.000000000000000000 ) ) ;
#83895=CARTESIAN_POINT ( 'NONE',  ( -12.04999999999999716, 2.500000000000000000, -6.495190528383298911 ) ) ;
#83896=FACE_OUTER_BOUND ( 'NONE', #121103, .T. ) ;
#83898=FACE_OUTER_BOUND ( 'NONE', #27068, .T. ) ;
#83899=FACE_OUTER_BOUND ( 'NONE', #22463, .T. ) ;
#83900=EDGE_CURVE ( 'NONE', #53205, #53076, #105936, .T. ) ;
#83901=EDGE_LOOP ( 'NONE', ( #33139, #87545, #65899, #87384 ) ) ;
#83902=ORIENTED_EDGE ( 'NONE', *, *, #49453, .F. ) ;
#83903=ORIENTED_EDGE ( 'NONE', *, *, #46181, .T. ) ;
#83904=DIRECTION ( 'NONE',  ( -0.000000000000000000, 1.000000000000000000, -0.000000000000000000 ) ) ;
#83905=ORIENTED_EDGE ( 'NONE', *, *, #17314, .T. ) ;
#83906=AXIS2_PLACEMENT_3D ( 'NONE', #106805, #59010, #117252 ) ;
#83907=AXIS2_PLACEMENT_3D ( 'NONE', #18585, #98413, #67016 ) ;
#83908=ORIENTED_EDGE ( 'NONE', *, *, #110867, .F. ) ;
#83909=ORIENTED_EDGE ( 'NONE', *, *, #91763, .F. ) ;
#83910=ORIENTED_EDGE ( 'NONE', *, *, #101432, .T. ) ;
#83911=DIRECTION ( 'NONE',  ( 0.000000000000000000, 1.000000000000000000, 0.000000000000000000 ) ) ;
#83912=CIRCLE ( 'NONE', #44202, 0.06509327318403745899 ) ;
#83913=LINE ( 'NONE', #94379, #57289 ) ;
#83914=AXIS2_PLACEMENT_3D ( 'NONE', #109015, #17408, #76996 ) ;
#83915=CARTESIAN_POINT ( 'NONE',  ( 6.449999999999931788, 12.50000000000000000, -2.511473670974877948 ) ) ;
#83916=DIRECTION ( 'NONE',  ( 0.000000000000000000, 1.000000000000000000, 0.000000000000000000 ) ) ;
#83917=VECTOR ( 'NONE', #114200, 1000.000000000000000 ) ;
#83918=CARTESIAN_POINT ( 'NONE',  ( 2.949999999999946887, 2.500000000000000000, -2.065063509461102065 ) ) ;
#83919=ORIENTED_EDGE ( 'NONE', *, *, #85901, .T. ) ;
#83920=DIRECTION ( 'NONE',  ( 0.000000000000000000, -0.9999939076577903929, 0.003490651415223739937 ) ) ;
#83921=ORIENTED_EDGE ( 'NONE', *, *, #4222, .T. ) ;
#83922=ORIENTED_EDGE ( 'NONE', *, *, #36838, .F. ) ;
#83923=ORIENTED_EDGE ( 'NONE', *, *, #35316, .T. ) ;
#83924=PLANE ( 'NONE',  #54712 ) ;
#83925=VERTEX_POINT ( 'NONE', #84396 ) ;
#83927=ORIENTED_EDGE ( 'NONE', *, *, #99841, .T. ) ;
#83928=DIRECTION ( 'NONE',  ( 0.000000000000000000, 1.000000000000000000, 0.000000000000000000 ) ) ;
#83929=ADVANCED_FACE ( 'NONE', ( #83126 ), #97517, .T. ) ;
#83930=DIRECTION ( 'NONE',  ( -0.000000000000000000, 1.000000000000000000, -0.000000000000000000 ) ) ;
#83931=DIRECTION ( 'NONE',  ( 0.000000000000000000, 0.000000000000000000, -1.000000000000000000 ) ) ;
#83932=FACE_OUTER_BOUND ( 'NONE', #74767, .T. ) ;
#83933=FACE_OUTER_BOUND ( 'NONE', #94130, .T. ) ;
#83934=DIRECTION ( 'NONE',  ( 0.000000000000000000, 1.000000000000000000, 0.000000000000000000 ) ) ;
#83935=DIRECTION ( 'NONE',  ( 0.000000000000000000, -0.000000000000000000, 1.000000000000000000 ) ) ;
#83936=AXIS2_PLACEMENT_3D ( 'NONE', #117592, #115680, #127452 ) ;
#83937=ADVANCED_FACE ( 'NONE', ( #34679 ), #18100, .T. ) ;
#83938=CONICAL_SURFACE ( 'NONE', #92253, 0.09999999999999982514, 0.003490658503988666988 ) ;
#83939=ORIENTED_EDGE ( 'NONE', *, *, #90739, .F. ) ;
#83940=DIRECTION ( 'NONE',  ( -4.274815082592931898E-19, -0.9999939076577903929, -0.003490651415223739937 ) ) ;
#83941=ORIENTED_EDGE ( 'NONE', *, *, #110104, .F. ) ;
#83942=DIRECTION ( 'NONE',  ( 0.000000000000000000, 0.000000000000000000, 1.000000000000000000 ) ) ;
#83943=ORIENTED_EDGE ( 'NONE', *, *, #11403, .T. ) ;
#83944=EDGE_CURVE ( 'NONE', #114247, #39021, #70335, .T. ) ;
#83945=ADVANCED_FACE ( 'NONE', ( #123657 ), #106030, .T. ) ;
#83946=EDGE_LOOP ( 'NONE', ( #48911, #120788 ) ) ;
#83947=CONICAL_SURFACE ( 'NONE', #71420, 0.09999999999999982514, 0.003490658503988666988 ) ;
#83948=CARTESIAN_POINT ( 'NONE',  ( 12.29999999999990479, 2.500000000000000000, 4.776537180435972196 ) ) ;
#83949=DIRECTION ( 'NONE',  ( 0.000000000000000000, 1.000000000000000000, 0.000000000000000000 ) ) ;
#83950=CONICAL_SURFACE ( 'NONE', #111128, 0.1000000000000000056, 0.003490658503988666988 ) ;
#83952=EDGE_CURVE ( 'NONE', #74899, #11954, #45398, .T. ) ;
#83953=CARTESIAN_POINT ( 'NONE',  ( -7.100000000000013856, 2.500000000000000000, 3.637306695894644726 ) ) ;
#83954=ORIENTED_EDGE ( 'NONE', *, *, #52785, .T. ) ;
#83955=ORIENTED_EDGE ( 'NONE', *, *, #54688, .T. ) ;
#83956=CARTESIAN_POINT ( 'NONE',  ( -7.950000000000016165, 2.500000000000000000, -6.495190528383297135 ) ) ;
#83958=ADVANCED_FACE ( 'NONE', ( #55587 ), #28674, .T. ) ;
#83959=CARTESIAN_POINT ( 'NONE',  ( 4.349999999999939249, 12.50000000000000000, 2.576566944158910744 ) ) ;
#83960=DIRECTION ( 'NONE',  ( 0.000000000000000000, 1.000000000000000000, 0.000000000000000000 ) ) ;
#83963=PLANE ( 'NONE',  #79316 ) ;
#83964=VERTEX_POINT ( 'NONE', #13710 ) ;
#83965=AXIS2_PLACEMENT_3D ( 'NONE', #122160, #83520, #123418 ) ;
#83966=VECTOR ( 'NONE', #49429, 1000.000000000000000 ) ;
#83967=ORIENTED_EDGE ( 'NONE', *, *, #76880, .T. ) ;
#83968=CARTESIAN_POINT ( 'NONE',  ( 6.049999999999934097, 2.500000000000000000, -6.148780366869526226 ) ) ;
#83969=DIRECTION ( 'NONE',  ( 0.000000000000000000, 0.000000000000000000, -1.000000000000000000 ) ) ;
#83970=AXIS2_PLACEMENT_3D ( 'NONE', #74066, #34148, #106103 ) ;
#83971=VECTOR ( 'NONE', #23914, 1000.000000000000000 ) ;
#83973=DIRECTION ( 'NONE',  ( 0.000000000000000000, 0.000000000000000000, 1.000000000000000000 ) ) ;
#83974=CARTESIAN_POINT ( 'NONE',  ( -12.69999999999999396, 2.500000000000000000, 0.3464101615137776813 ) ) ;
#83975=DIRECTION ( 'NONE',  ( 0.000000000000000000, -0.9999939076577903929, 0.003490651415223739937 ) ) ;
#83976=CARTESIAN_POINT ( 'NONE',  ( -9.550000000000002487, 2.500000000000000000, 6.495190528383297135 ) ) ;
#83977=ORIENTED_EDGE ( 'NONE', *, *, #44271, .F. ) ;
#83978=DIRECTION ( 'NONE',  ( 0.000000000000000000, 0.000000000000000000, 1.000000000000000000 ) ) ;
#83979=ADVANCED_FACE ( 'NONE', ( #23541 ), #85091, .T. ) ;
#83980=CARTESIAN_POINT ( 'NONE',  ( 5.599999999999931255, 12.50000000000000000, 4.048810130592458201 ) ) ;
#83981=CARTESIAN_POINT ( 'NONE',  ( -6.450000000000017941, 2.500000000000000000, -6.841600689897077814 ) ) ;
#83982=ORIENTED_EDGE ( 'NONE', *, *, #86480, .T. ) ;
#83983=ADVANCED_FACE ( 'NONE', ( #16282 ), #83057, .T. ) ;
#83984=EDGE_CURVE ( 'NONE', #84019, #109827, #22430, .T. ) ;
#83985=DIRECTION ( 'NONE',  ( 0.000000000000000000, 0.000000000000000000, 1.000000000000000000 ) ) ;
#83986=ORIENTED_EDGE ( 'NONE', *, *, #127278, .F. ) ;
#83987=CARTESIAN_POINT ( 'NONE',  ( -11.84999999999999787, 2.500000000000000000, -6.148780366869522673 ) ) ;
#83988=CIRCLE ( 'NONE', #23346, 0.06509327318403745899 ) ;
#83989=CONICAL_SURFACE ( 'NONE', #29624, 0.1000000000000002554, 0.003490658503988666988 ) ;
#83990=ADVANCED_FACE ( 'NONE', ( #28713 ), #5657, .T. ) ;
#83991=AXIS2_PLACEMENT_3D ( 'NONE', #116620, #68815, #46593 ) ;
#83992=ORIENTED_EDGE ( 'NONE', *, *, #16280, .T. ) ;
#83993=DIRECTION ( 'NONE',  ( 0.000000000000000000, -0.9999939076577903929, 0.003490651415223739937 ) ) ;
#83994=DIRECTION ( 'NONE',  ( 0.000000000000000000, 0.000000000000000000, 1.000000000000000000 ) ) ;
#83995=EDGE_CURVE ( 'NONE', #80322, #97094, #98081, .T. ) ;
#83996=DIRECTION ( 'NONE',  ( 0.000000000000000000, 0.000000000000000000, 1.000000000000000000 ) ) ;
#83997=ADVANCED_FACE ( 'NONE', ( #107903 ), #26609, .T. ) ;
#83998=ORIENTED_EDGE ( 'NONE', *, *, #45936, .F. ) ;
#83999=VECTOR ( 'NONE', #4443, 1000.000000000000000 ) ;
#84000=CARTESIAN_POINT ( 'NONE',  ( 13.09999999999989839, 12.50000000000000000, -0.2813168883297409439 ) ) ;
#84001=AXIS2_PLACEMENT_3D ( 'NONE', #52691, #40308, #80228 ) ;
#84002=EDGE_CURVE ( 'NONE', #21282, #129137, #6443, .T. ) ;
#84003=CARTESIAN_POINT ( 'NONE',  ( 11.64999999999990266, 12.50000000000000000, 2.165063509461097713 ) ) ;
#84004=AXIS2_PLACEMENT_3D ( 'NONE', #99211, #46886, #126732 ) ;
#84005=AXIS2_PLACEMENT_3D ( 'NONE', #97678, #124573, #125210 ) ;
#84006=VERTEX_POINT ( 'NONE', #127550 ) ;
#84008=AXIS2_PLACEMENT_3D ( 'NONE', #35124, #123470, #63925 ) ;
#84009=CARTESIAN_POINT ( 'NONE',  ( 4.199999999999938005, 2.500000000000000000, 4.330127018922196314 ) ) ;
#84010=EDGE_CURVE ( 'NONE', #58932, #70277, #27390, .T. ) ;
#84011=ORIENTED_EDGE ( 'NONE', *, *, #82460, .F. ) ;
#84012=ORIENTED_EDGE ( 'NONE', *, *, #94342, .F. ) ;
#84013=CARTESIAN_POINT ( 'NONE',  ( 13.09999999999989839, 12.50000000000000000, 0.3464101615137735735 ) ) ;
#84014=CARTESIAN_POINT ( 'NONE',  ( 8.949999999999921130, 2.500000000000000000, -6.741600689897078169 ) ) ;
#84015=CARTESIAN_POINT ( 'NONE',  ( 2.699999999999947331, 2.500000000000000000, -0.3464101615137783474 ) ) ;
#84016=ORIENTED_EDGE ( 'NONE', *, *, #44377, .F. ) ;
#84017=CARTESIAN_POINT ( 'NONE',  ( -4.400000000000028777, 2.500000000000000000, -3.983716857408426293 ) ) ;
#84018=DIRECTION ( 'NONE',  ( -0.000000000000000000, 1.000000000000000000, -0.000000000000000000 ) ) ;
#84019=VERTEX_POINT ( 'NONE', #47066 ) ;
#84020=DIRECTION ( 'NONE',  ( 0.000000000000000000, 1.000000000000000000, 0.000000000000000000 ) ) ;
#84021=DIRECTION ( 'NONE',  ( 0.000000000000000000, 1.000000000000000000, 0.000000000000000000 ) ) ;
#84022=DIRECTION ( 'NONE',  ( 0.000000000000000000, -0.000000000000000000, 1.000000000000000000 ) ) ;
#84023=CARTESIAN_POINT ( 'NONE',  ( -1.450000000000035927, 2.500000000000000000, -6.048780366869526581 ) ) ;
#84024=DIRECTION ( 'NONE',  ( 0.000000000000000000, 1.000000000000000000, 0.000000000000000000 ) ) ;
#84025=CARTESIAN_POINT ( 'NONE',  ( 5.399999999999931966, 12.50000000000000000, 4.330127018922196314 ) ) ;
#84026=PLANE ( 'NONE',  #94261 ) ;
#84027=CIRCLE ( 'NONE', #27588, 0.06509327318403745899 ) ;
#84028=AXIS2_PLACEMENT_3D ( 'NONE', #95072, #45336, #85245 ) ;
#84029=EDGE_LOOP ( 'NONE', ( #121406, #45110 ) ) ;
#84031=EDGE_LOOP ( 'NONE', ( #98718, #64803 ) ) ;
#84032=ORIENTED_EDGE ( 'NONE', *, *, #104492, .F. ) ;
#84033=CARTESIAN_POINT ( 'NONE',  ( -11.44999999999999751, 12.50000000000000000, 6.841600689897072485 ) ) ;
#84035=CARTESIAN_POINT ( 'NONE',  ( -12.29999999999999538, 2.500000000000000000, 4.776537180435972196 ) ) ;
#84036=ORIENTED_EDGE ( 'NONE', *, *, #28397, .T. ) ;
#84037=FACE_BOUND ( 'NONE', #128590, .T. ) ;
#84038=VECTOR ( 'NONE', #14907, 1000.000000000000000 ) ;
#84039=DIRECTION ( 'NONE',  ( 0.000000000000000000, 0.000000000000000000, 1.000000000000000000 ) ) ;
#84040=DIRECTION ( 'NONE',  ( -0.000000000000000000, 1.000000000000000000, -0.000000000000000000 ) ) ;
#84041=AXIS2_PLACEMENT_3D ( 'NONE', #42913, #20675, #69765 ) ;
#84042=AXIS2_PLACEMENT_3D ( 'NONE', #41493, #113426, #21841 ) ;
#84043=CARTESIAN_POINT ( 'NONE',  ( -6.850000000000013856, 12.50000000000000000, 2.446380397790835826 ) ) ;
#84044=AXIS2_PLACEMENT_3D ( 'NONE', #92672, #13454, #3644 ) ;
#84045=EDGE_CURVE ( 'NONE', #98668, #47201, #93417, .T. ) ;
#84046=DIRECTION ( 'NONE',  ( -0.000000000000000000, 1.000000000000000000, -0.000000000000000000 ) ) ;
#84047=CARTESIAN_POINT ( 'NONE',  ( -2.500000000000030642, 12.50000000000000000, -5.022947341949754119 ) ) ;
#84048=DIRECTION ( 'NONE',  ( 0.000000000000000000, 1.000000000000000000, 0.000000000000000000 ) ) ;
#84049=CARTESIAN_POINT ( 'NONE',  ( 4.399999999999939071, 12.50000000000000000, -0.3464101615137782364 ) ) ;
#84050=CARTESIAN_POINT ( 'NONE',  ( -3.150000000000029221, 2.500000000000000000, -1.818653347947326138 ) ) ;
#84051=CARTESIAN_POINT ( 'NONE',  ( 5.849999999999933920, 2.500000000000000000, 5.702370205355745014 ) ) ;
#84052=CONICAL_SURFACE ( 'NONE', #61084, 0.1000000000000002554, 0.003490658503988666988 ) ;
#84053=DIRECTION ( 'NONE',  ( -4.274815082592931898E-19, -0.9999939076577903929, -0.003490651415223739937 ) ) ;
#84054=VERTEX_POINT ( 'NONE', #37250 ) ;
#84055=CIRCLE ( 'NONE', #127976, 0.06509327318403745899 ) ;
#84056=ADVANCED_FACE ( 'NONE', ( #58812 ), #67970, .T. ) ;
#84057=ORIENTED_EDGE ( 'NONE', *, *, #1246, .F. ) ;
#84058=EDGE_LOOP ( 'NONE', ( #107655, #77339, #92101, #92248 ) ) ;
#84060=CIRCLE ( 'NONE', #102828, 0.06509327318403745899 ) ;
#84061=ORIENTED_EDGE ( 'NONE', *, *, #102573, .T. ) ;
#84062=AXIS2_PLACEMENT_3D ( 'NONE', #8575, #87788, #6626 ) ;
#84063=CIRCLE ( 'NONE', #113307, 0.06509327318403745899 ) ;
#84064=ORIENTED_EDGE ( 'NONE', *, *, #4510, .T. ) ;
#84065=DIRECTION ( 'NONE',  ( 0.000000000000000000, -0.9999939076577903929, 0.003490651415223739937 ) ) ;
#84066=VERTEX_POINT ( 'NONE', #76521 ) ;
#84067=VERTEX_POINT ( 'NONE', #117700 ) ;
#84068=VECTOR ( 'NONE', #48449, 1000.000000000000000 ) ;
#84069=VECTOR ( 'NONE', #84529, 1000.000000000000000 ) ;
#84070=FACE_OUTER_BOUND ( 'NONE', #86404, .T. ) ;
#84071=DIRECTION ( 'NONE',  ( 0.000000000000000000, 0.000000000000000000, -1.000000000000000000 ) ) ;
#84072=DIRECTION ( 'NONE',  ( -0.000000000000000000, 1.000000000000000000, -0.000000000000000000 ) ) ;
#84073=DIRECTION ( 'NONE',  ( 0.000000000000000000, -0.000000000000000000, 1.000000000000000000 ) ) ;
#84074=ORIENTED_EDGE ( 'NONE', *, *, #21618, .F. ) ;
#84075=DIRECTION ( 'NONE',  ( 0.000000000000000000, -0.000000000000000000, 1.000000000000000000 ) ) ;
#84076=ORIENTED_EDGE ( 'NONE', *, *, #93874, .T. ) ;
#84077=ORIENTED_EDGE ( 'NONE', *, *, #74794, .F. ) ;
#84078=DIRECTION ( 'NONE',  ( 0.000000000000000000, -0.000000000000000000, 1.000000000000000000 ) ) ;
#84079=VERTEX_POINT ( 'NONE', #86974 ) ;
#84080=DIRECTION ( 'NONE',  ( 0.000000000000000000, -0.000000000000000000, 1.000000000000000000 ) ) ;
#84081=ORIENTED_EDGE ( 'NONE', *, *, #70830, .T. ) ;
#84082=VERTEX_POINT ( 'NONE', #77160 ) ;
#84083=CARTESIAN_POINT ( 'NONE',  ( -12.09999999999999609, 12.50000000000000000, -0.6928203230275501445 ) ) ;
#84084=DIRECTION ( 'NONE',  ( 0.000000000000000000, 0.000000000000000000, 1.000000000000000000 ) ) ;
#84085=DIRECTION ( 'NONE',  ( -0.000000000000000000, 1.000000000000000000, -0.000000000000000000 ) ) ;
#84087=CARTESIAN_POINT ( 'NONE',  ( -1.850000000000033840, 12.50000000000000000, 2.511473670974873507 ) ) ;
#84088=AXIS2_PLACEMENT_3D ( 'NONE', #129109, #78707, #19777 ) ;
#84089=CARTESIAN_POINT ( 'NONE',  ( -10.60000000000000142, 12.50000000000000000, -0.3464101615137782364 ) ) ;
#84090=ORIENTED_EDGE ( 'NONE', *, *, #57255, .T. ) ;
#84091=CARTESIAN_POINT ( 'NONE',  ( -8.950000000000004619, 2.500000000000000000, 6.148780366869520897 ) ) ;
#84092=ADVANCED_FACE ( 'NONE', ( #9055 ), #76694, .T. ) ;
#84094=ORIENTED_EDGE ( 'NONE', *, *, #88795, .T. ) ;
#84095=CARTESIAN_POINT ( 'NONE',  ( 17.50000000000000000, 2.499999999999999556, -3.666666666666662522 ) ) ;
#84096=AXIS2_PLACEMENT_3D ( 'NONE', #70728, #10503, #119826 ) ;
#84097=EDGE_LOOP ( 'NONE', ( #84057, #29794 ) ) ;
#84098=DIRECTION ( 'NONE',  ( -0.000000000000000000, -1.000000000000000000, -0.000000000000000000 ) ) ;
#84099=DIRECTION ( 'NONE',  ( 0.000000000000000000, 1.000000000000000000, 0.000000000000000000 ) ) ;
#84100=CIRCLE ( 'NONE', #61126, 0.06509327318403745899 ) ;
#84101=AXIS2_PLACEMENT_3D ( 'NONE', #119666, #58825, #49667 ) ;
#84102=CARTESIAN_POINT ( 'NONE',  ( -7.050000000000013145, 12.50000000000000000, 2.165063509461097713 ) ) ;
#84103=EDGE_CURVE ( 'NONE', #66863, #57597, #122756, .T. ) ;
#84104=CARTESIAN_POINT ( 'NONE',  ( -8.749999999999971578, 2.500000000000000000, 6.395190528383296602 ) ) ;
#84105=EDGE_CURVE ( 'NONE', #35498, #22187, #21858, .T. ) ;
#84106=ORIENTED_EDGE ( 'NONE', *, *, #27520, .F. ) ;
#84107=AXIS2_PLACEMENT_3D ( 'NONE', #11671, #101356, #42438 ) ;
#84108=EDGE_CURVE ( 'NONE', #77492, #78495, #74630, .T. ) ;
#84109=DIRECTION ( 'NONE',  ( 0.000000000000000000, 0.000000000000000000, -1.000000000000000000 ) ) ;
#84110=ORIENTED_EDGE ( 'NONE', *, *, #69111, .T. ) ;
#84112=VERTEX_POINT ( 'NONE', #70553 ) ;
#84113=EDGE_LOOP ( 'NONE', ( #60895, #90914, #82855, #52062 ) ) ;
#84114=DIRECTION ( 'NONE',  ( -0.000000000000000000, -1.000000000000000000, -0.000000000000000000 ) ) ;
#84115=DIRECTION ( 'NONE',  ( 0.000000000000000000, 0.000000000000000000, 1.000000000000000000 ) ) ;
#84116=EDGE_CURVE ( 'NONE', #122938, #39770, #36986, .T. ) ;
#84118=LINE ( 'NONE', #16654, #40848 ) ;
#84119=AXIS2_PLACEMENT_3D ( 'NONE', #16826, #128779, #78381 ) ;
#84120=CARTESIAN_POINT ( 'NONE',  ( 4.349999999999940137, 2.500000000000000000, -2.511473670974877948 ) ) ;
#84121=DIRECTION ( 'NONE',  ( -0.000000000000000000, -1.000000000000000000, -0.000000000000000000 ) ) ;
#84122=AXIS2_PLACEMENT_3D ( 'NONE', #101051, #129256, #29112 ) ;
#84123=ORIENTED_EDGE ( 'NONE', *, *, #80631, .F. ) ;
#84124=CARTESIAN_POINT ( 'NONE',  ( 9.599999999999914380, 2.500000000000000000, -3.537306695894649966 ) ) ;
#84125=EDGE_LOOP ( 'NONE', ( #105632, #80026 ) ) ;
#84126=CARTESIAN_POINT ( 'NONE',  ( 4.799999999999937650, 12.50000000000000000, -0.2813168883297408329 ) ) ;
#84127=CARTESIAN_POINT ( 'NONE',  ( 4.999999999999933387, 2.500000000000000000, 5.022947341949748790 ) ) ;
#84128=DIRECTION ( 'NONE',  ( 0.000000000000000000, 1.000000000000000000, 0.000000000000000000 ) ) ;
#84129=AXIS2_PLACEMENT_3D ( 'NONE', #108946, #97213, #76933 ) ;
#84130=VECTOR ( 'NONE', #69606, 1000.000000000000000 ) ;
#84131=ORIENTED_EDGE ( 'NONE', *, *, #127711, .F. ) ;
#84132=CONICAL_SURFACE ( 'NONE', #10958, 0.1000000000000002554, 0.003490658503988666988 ) ;
#84133=DIRECTION ( 'NONE',  ( -4.274815082592931898E-19, -0.9999939076577903929, -0.003490651415223739937 ) ) ;
#84135=CIRCLE ( 'NONE', #6849, 0.06509327318403745899 ) ;
#84136=VERTEX_POINT ( 'NONE', #121580 ) ;
#84137=FACE_OUTER_BOUND ( 'NONE', #18325, .T. ) ;
#84138=AXIS2_PLACEMENT_3D ( 'NONE', #7222, #98197, #77274 ) ;
#84139=VERTEX_POINT ( 'NONE', #41767 ) ;
#84140=AXIS2_PLACEMENT_3D ( 'NONE', #15002, #36629, #16299 ) ;
#84141=AXIS2_PLACEMENT_3D ( 'NONE', #1991, #100208, #72043 ) ;
#84142=ORIENTED_EDGE ( 'NONE', *, *, #86763, .F. ) ;
#84143=VECTOR ( 'NONE', #49165, 1000.000000000000000 ) ;
#84144=CARTESIAN_POINT ( 'NONE',  ( -12.89999999999999147, 2.500000000000000000, 4.922947341949748257 ) ) ;
#84145=ADVANCED_FACE ( 'NONE', ( #62042 ), #49651, .T. ) ;
#84146=EDGE_CURVE ( 'NONE', #24096, #64597, #20820, .T. ) ;
#84147=CONICAL_SURFACE ( 'NONE', #86201, 0.1000000000000002554, 0.003490658503988666988 ) ;
#84148=ORIENTED_EDGE ( 'NONE', *, *, #64388, .T. ) ;
#84149=PLANE ( 'NONE',  #40522 ) ;
#84150=DIRECTION ( 'NONE',  ( 0.000000000000000000, 1.000000000000000000, 0.000000000000000000 ) ) ;
#84151=EDGE_CURVE ( 'NONE', #27897, #83521, #1172, .T. ) ;
#84152=FACE_OUTER_BOUND ( 'NONE', #2221, .T. ) ;
#84153=EDGE_LOOP ( 'NONE', ( #69226, #42655, #15970, #119342 ) ) ;
#84154=AXIS2_PLACEMENT_3D ( 'NONE', #91615, #2570, #1935 ) ;
#84155=ADVANCED_FACE ( 'NONE', ( #71861 ), #11932, .T. ) ;
#84156=CARTESIAN_POINT ( 'NONE',  ( 3.349999999999944578, 12.50000000000000000, -5.802370205355749988 ) ) ;
#84157=DIRECTION ( 'NONE',  ( 0.000000000000000000, 0.000000000000000000, 1.000000000000000000 ) ) ;
#84158=ORIENTED_EDGE ( 'NONE', *, *, #37959, .F. ) ;
#84159=ADVANCED_FACE ( 'NONE', ( #100648 ), #64161, .T. ) ;
#84160=CARTESIAN_POINT ( 'NONE',  ( -3.750000000000027534, 2.500000000000000000, 2.957883832488649389 ) ) ;
#84161=CARTESIAN_POINT ( 'NONE',  ( 1.449999999999950440, 12.50000000000000000, 6.083687093685482772 ) ) ;
#84162=ORIENTED_EDGE ( 'NONE', *, *, #3509, .F. ) ;
#84163=EDGE_CURVE ( 'NONE', #60727, #18083, #89302, .T. ) ;
#84164=EDGE_CURVE ( 'NONE', #63903, #32296, #9887, .T. ) ;
#84165=EDGE_LOOP ( 'NONE', ( #109699, #81108, #95973, #19312 ) ) ;
#84166=VERTEX_POINT ( 'NONE', #10348 ) ;
#84167=DIRECTION ( 'NONE',  ( 0.000000000000000000, 1.000000000000000000, 0.000000000000000000 ) ) ;
#84168=LINE ( 'NONE', #44244, #85470 ) ;
#84169=DIRECTION ( 'NONE',  ( -0.000000000000000000, 1.000000000000000000, -0.000000000000000000 ) ) ;
#84170=FACE_BOUND ( 'NONE', #33700, .T. ) ;
#84171=ORIENTED_EDGE ( 'NONE', *, *, #83379, .T. ) ;
#84173=ADVANCED_FACE ( 'NONE', ( #111781 ), #22131, .T. ) ;
#84174=DIRECTION ( 'NONE',  ( 0.000000000000000000, 0.000000000000000000, 1.000000000000000000 ) ) ;
#84175=CARTESIAN_POINT ( 'NONE',  ( -14.59999999999998366, 2.500000000000000000, 0.6928203230275518099 ) ) ;
#84176=CIRCLE ( 'NONE', #27746, 0.06509327318403741736 ) ;
#84177=AXIS2_PLACEMENT_3D ( 'NONE', #61549, #111251, #21615 ) ;
#84178=DIRECTION ( 'NONE',  ( 0.000000000000000000, 0.000000000000000000, -1.000000000000000000 ) ) ;
#84179=AXIS2_PLACEMENT_3D ( 'NONE', #94252, #123079, #82523 ) ;
#84180=FACE_OUTER_BOUND ( 'NONE', #123144, .T. ) ;
#84181=DIRECTION ( 'NONE',  ( 0.000000000000000000, 0.000000000000000000, 1.000000000000000000 ) ) ;
#84183=CIRCLE ( 'NONE', #73715, 0.1000000000000000472 ) ;
#84185=ORIENTED_EDGE ( 'NONE', *, *, #3558, .T. ) ;
#84186=EDGE_LOOP ( 'NONE', ( #28183, #46230, #18439, #55001 ) ) ;
#84187=ORIENTED_EDGE ( 'NONE', *, *, #62145, .F. ) ;
#84188=VERTEX_POINT ( 'NONE', #79109 ) ;
#84189=CIRCLE ( 'NONE', #75781, 0.1000000000000002554 ) ;
#84190=EDGE_LOOP ( 'NONE', ( #27063, #10029 ) ) ;
#84191=LINE ( 'NONE', #114304, #21320 ) ;
#84192=CIRCLE ( 'NONE', #126050, 0.06509327318403745899 ) ;
#84193=CONICAL_SURFACE ( 'NONE', #27763, 0.09999999999999982514, 0.003490658503988666988 ) ;
#84194=FACE_OUTER_BOUND ( 'NONE', #75987, .T. ) ;
#84195=ORIENTED_EDGE ( 'NONE', *, *, #108221, .T. ) ;
#84196=FACE_BOUND ( 'NONE', #36, .T. ) ;
#84197=CARTESIAN_POINT ( 'NONE',  ( -3.350000000000031619, 2.500000000000000000, -7.288010851410854585 ) ) ;
#84198=CARTESIAN_POINT ( 'NONE',  ( 6.449999999999928235, 2.500000000000000000, 2.411473670974873862 ) ) ;
#84199=ORIENTED_EDGE ( 'NONE', *, *, #88894, .T. ) ;
#84200=DIRECTION ( 'NONE',  ( 0.000000000000000000, -0.000000000000000000, 1.000000000000000000 ) ) ;
#84201=DIRECTION ( 'NONE',  ( 0.000000000000000000, 0.000000000000000000, 1.000000000000000000 ) ) ;
#84202=CARTESIAN_POINT ( 'NONE',  ( 4.799999999999935874, 2.500000000000000000, 0.2464101615137735679 ) ) ;
#84203=ORIENTED_EDGE ( 'NONE', *, *, #64785, .F. ) ;
#84204=DIRECTION ( 'NONE',  ( 0.000000000000000000, 0.000000000000000000, 1.000000000000000000 ) ) ;
#84205=AXIS2_PLACEMENT_3D ( 'NONE', #91254, #109613, #61150 ) ;
#84206=ORIENTED_EDGE ( 'NONE', *, *, #117667, .T. ) ;
#84207=EDGE_CURVE ( 'NONE', #37050, #40175, #59487, .T. ) ;
#84208=EDGE_LOOP ( 'NONE', ( #46405, #80934, #154, #17669 ) ) ;
#84209=VERTEX_POINT ( 'NONE', #99387 ) ;
#84210=DIRECTION ( 'NONE',  ( 0.000000000000000000, 0.000000000000000000, 1.000000000000000000 ) ) ;
#84211=CARTESIAN_POINT ( 'NONE',  ( -11.04999999999999893, 2.500000000000000000, 1.918653347947321564 ) ) ;
#84212=CARTESIAN_POINT ( 'NONE',  ( -3.950000000000025491, 12.50000000000000000, 6.213873640053559022 ) ) ;
#84213=ORIENTED_EDGE ( 'NONE', *, *, #34960, .T. ) ;
#84214=FACE_OUTER_BOUND ( 'NONE', #64652, .T. ) ;
#84215=AXIS2_PLACEMENT_3D ( 'NONE', #107704, #58612, #87398 ) ;
#84216=DIRECTION ( 'NONE',  ( -0.000000000000000000, 1.000000000000000000, -0.000000000000000000 ) ) ;
#84217=FACE_OUTER_BOUND ( 'NONE', #91806, .T. ) ;
#84218=FACE_OUTER_BOUND ( 'NONE', #56129, .T. ) ;
#84219=ORIENTED_EDGE ( 'NONE', *, *, #117121, .F. ) ;
#84220=LINE ( 'NONE', #34515, #22411 ) ;
#84221=AXIS2_PLACEMENT_3D ( 'NONE', #120720, #113311, #124430 ) ;
#84222=ORIENTED_EDGE ( 'NONE', *, *, #98279, .T. ) ;
#84223=CARTESIAN_POINT ( 'NONE',  ( 8.349999999999919709, 2.500000000000000000, -2.065063509461102065 ) ) ;
#84224=AXIS2_PLACEMENT_3D ( 'NONE', #5374, #94395, #85231 ) ;
#84225=ORIENTED_EDGE ( 'NONE', *, *, #30986, .T. ) ;
#84226=AXIS2_PLACEMENT_3D ( 'NONE', #747, #79338, #28292 ) ;
#84227=VERTEX_POINT ( 'NONE', #129513 ) ;
#84228=CARTESIAN_POINT ( 'NONE',  ( 3.349999999999942801, 12.50000000000000000, 2.922977105672686982 ) ) ;
#84229=DIRECTION ( 'NONE',  ( 0.000000000000000000, 1.000000000000000000, 0.000000000000000000 ) ) ;
#84230=DIRECTION ( 'NONE',  ( 0.000000000000000000, 0.000000000000000000, 1.000000000000000000 ) ) ;
#84231=DIRECTION ( 'NONE',  ( -4.274815082592931898E-19, -0.9999939076577903929, -0.003490651415223739937 ) ) ;
#84233=CIRCLE ( 'NONE', #88136, 0.06509327318403745899 ) ;
#84234=ORIENTED_EDGE ( 'NONE', *, *, #80522, .T. ) ;
#84235=EDGE_LOOP ( 'NONE', ( #34574, #105885, #70908, #53736 ) ) ;
#84236=AXIS2_PLACEMENT_3D ( 'NONE', #88802, #87497, #128757 ) ;
#84237=CARTESIAN_POINT ( 'NONE',  ( 11.64999999999990621, 2.500000000000000000, -2.265063509461101798 ) ) ;
#84238=CARTESIAN_POINT ( 'NONE',  ( 76.44225496929378494, 3.905139198807624723, -5.869654418954768360 ) ) ;
#84239=AXIS2_PLACEMENT_3D ( 'NONE', #128225, #78489, #118383 ) ;
#84240=CIRCLE ( 'NONE', #67504, 0.06509327318403745899 ) ;
#84241=CIRCLE ( 'NONE', #123950, 0.06509327318403745899 ) ;
#84242=DIRECTION ( 'NONE',  ( 0.000000000000000000, -0.9999939076577903929, 0.003490651415223739937 ) ) ;
#84243=VERTEX_POINT ( 'NONE', #39835 ) ;
#84244=VERTEX_POINT ( 'NONE', #90176 ) ;
#84245=CARTESIAN_POINT ( 'NONE',  ( 4.349999999999941025, 2.500000000000000000, -6.048780366869526581 ) ) ;
#84246=AXIS2_PLACEMENT_3D ( 'NONE', #22727, #113016, #62647 ) ;
#84247=ORIENTED_EDGE ( 'NONE', *, *, #82821, .T. ) ;
#84248=DIRECTION ( 'NONE',  ( -0.000000000000000000, -1.000000000000000000, -0.000000000000000000 ) ) ;
#84249=EDGE_CURVE ( 'NONE', #108498, #67661, #20256, .T. ) ;
#84250=DIRECTION ( 'NONE',  ( -0.000000000000000000, -1.000000000000000000, -0.000000000000000000 ) ) ;
#84251=ORIENTED_EDGE ( 'NONE', *, *, #47028, .T. ) ;
#84252=AXIS2_PLACEMENT_3D ( 'NONE', #48318, #37848, #78447 ) ;
#84253=CARTESIAN_POINT ( 'NONE',  ( 7.049999999999926992, 2.500000000000000000, 2.065063509461097624 ) ) ;
#84254=DIRECTION ( 'NONE',  ( -0.000000000000000000, 1.000000000000000000, -0.000000000000000000 ) ) ;
#84255=CARTESIAN_POINT ( 'NONE',  ( 6.049999999999930544, 2.500000000000000000, 2.611473670974873151 ) ) ;
#84256=ADVANCED_FACE ( 'NONE', ( #109849 ), #7716, .T. ) ;
#84257=DIRECTION ( 'NONE',  ( 0.000000000000000000, 0.000000000000000000, -1.000000000000000000 ) ) ;
#84258=EDGE_CURVE ( 'NONE', #72199, #41083, #80394, .T. ) ;
#84259=ORIENTED_EDGE ( 'NONE', *, *, #32775, .T. ) ;
#84260=DIRECTION ( 'NONE',  ( 0.000000000000000000, 1.000000000000000000, 0.000000000000000000 ) ) ;
#84261=CARTESIAN_POINT ( 'NONE',  ( 32.15727368887977633, -2.842525632566917704, 4.549395963656282404 ) ) ;
#84263=ORIENTED_EDGE ( 'NONE', *, *, #121865, .T. ) ;
#84264=EDGE_CURVE ( 'NONE', #70303, #100605, #54774, .T. ) ;
#84265=ORIENTED_EDGE ( 'NONE', *, *, #4412, .T. ) ;
#84266=VECTOR ( 'NONE', #61579, 1000.000000000000000 ) ;
#84267=CIRCLE ( 'NONE', #52976, 0.1000000000000002554 ) ;
#84268=ADVANCED_FACE ( 'NONE', ( #92120 ), #22772, .T. ) ;
#84270=DIRECTION ( 'NONE',  ( -0.000000000000000000, 1.000000000000000000, -0.000000000000000000 ) ) ;
#84271=EDGE_CURVE ( 'NONE', #125100, #23084, #85189, .T. ) ;
#84272=ADVANCED_FACE ( 'NONE', ( #72507 ), #112429, .T. ) ;
#84273=CARTESIAN_POINT ( 'NONE',  ( -13.14999999999999147, 2.500000000000000000, 2.511473670974877503 ) ) ;
#84274=DIRECTION ( 'NONE',  ( 0.000000000000000000, 0.000000000000000000, 1.000000000000000000 ) ) ;
#84275=CARTESIAN_POINT ( 'NONE',  ( -2.300000000000032685, 12.50000000000000000, -4.741630453620016006 ) ) ;
#84276=CARTESIAN_POINT ( 'NONE',  ( -10.20000000000000462, 12.50000000000000000, -4.676537180435973440 ) ) ;
#84277=FACE_OUTER_BOUND ( 'NONE', #36703, .T. ) ;
#84278=CONICAL_SURFACE ( 'NONE', #123984, 0.1000000000000002554, 0.003490658503988666988 ) ;
#84279=DIRECTION ( 'NONE',  ( 0.000000000000000000, -0.000000000000000000, 1.000000000000000000 ) ) ;
#84280=DIRECTION ( 'NONE',  ( 0.000000000000000000, 0.000000000000000000, 1.000000000000000000 ) ) ;
#84281=DIRECTION ( 'NONE',  ( 0.000000000000000000, 1.000000000000000000, 0.000000000000000000 ) ) ;
#84282=AXIS2_PLACEMENT_3D ( 'NONE', #50021, #29089, #87961 ) ;
#84283=EDGE_CURVE ( 'NONE', #68896, #12189, #62223, .T. ) ;
#84284=PLANE ( 'NONE',  #22954 ) ;
#84285=VERTEX_POINT ( 'NONE', #65234 ) ;
#84286=CIRCLE ( 'NONE', #109323, 0.06509327318403745899 ) ;
#84287=VERTEX_POINT ( 'NONE', #82326 ) ;
#84288=AXIS2_PLACEMENT_3D ( 'NONE', #124876, #65940, #64659 ) ;
#84289=AXIS2_PLACEMENT_3D ( 'NONE', #23122, #120686, #70938 ) ;
#84290=ORIENTED_EDGE ( 'NONE', *, *, #38473, .F. ) ;
#84291=CIRCLE ( 'NONE', #98859, 0.1000000000000000472 ) ;
#84292=CIRCLE ( 'NONE', #21600, 0.06509327318403745899 ) ;
#84293=ORIENTED_EDGE ( 'NONE', *, *, #24651, .T. ) ;
#84294=LINE ( 'NONE', #21023, #83355 ) ;
#84295=DIRECTION ( 'NONE',  ( 0.000000000000000000, 1.000000000000000000, 0.000000000000000000 ) ) ;
#84296=DIRECTION ( 'NONE',  ( 0.000000000000000000, 1.000000000000000000, 0.000000000000000000 ) ) ;
#84297=VECTOR ( 'NONE', #51145, 1000.000000000000000 ) ;
#84298=ORIENTED_EDGE ( 'NONE', *, *, #6545, .T. ) ;
#84299=CARTESIAN_POINT ( 'NONE',  ( 13.34999999999990017, 12.50000000000000000, 2.857883832488649301 ) ) ;
#84300=DIRECTION ( 'NONE',  ( -0.000000000000000000, -1.000000000000000000, -0.000000000000000000 ) ) ;
#84301=LINE ( 'NONE', #105878, #14080 ) ;
#84302=EDGE_LOOP ( 'NONE', ( #63876, #19856 ) ) ;
#84303=DIRECTION ( 'NONE',  ( -0.000000000000000000, -1.000000000000000000, -0.000000000000000000 ) ) ;
#84304=AXIS2_PLACEMENT_3D ( 'NONE', #68227, #116045, #55204 ) ;
#84305=PLANE ( 'NONE',  #27058 ) ;
#84306=ORIENTED_EDGE ( 'NONE', *, *, #120346, .T. ) ;
#84307=VERTEX_POINT ( 'NONE', #14199 ) ;
#84308=VERTEX_POINT ( 'NONE', #12270 ) ;
#84309=VERTEX_POINT ( 'NONE', #122253 ) ;
#84310=DIRECTION ( 'NONE',  ( 0.000000000000000000, -0.9999939076577903929, 0.003490651415223739937 ) ) ;
#84311=ADVANCED_FACE ( 'NONE', ( #44315 ), #108161, .T. ) ;
#84312=CARTESIAN_POINT ( 'NONE',  ( -12.69999999999999041, 2.500000000000000000, 4.083716857408421497 ) ) ;
#84313=CONICAL_SURFACE ( 'NONE', #48830, 0.1000000000000000472, 0.003490658503988666988 ) ;
#84314=DIRECTION ( 'NONE',  ( 0.000000000000000000, 1.000000000000000000, 0.000000000000000000 ) ) ;
#84315=EDGE_CURVE ( 'NONE', #40907, #56932, #14829, .T. ) ;
#84316=VECTOR ( 'NONE', #93226, 1000.000000000000000 ) ;
#84317=CARTESIAN_POINT ( 'NONE',  ( -1.650000000000034328, 2.500000000000000000, -6.395190528383301931 ) ) ;
#84318=ORIENTED_EDGE ( 'NONE', *, *, #54396, .F. ) ;
#84319=ADVANCED_FACE ( 'NONE', ( #83614 ), #126963, .T. ) ;
#84320=DIRECTION ( 'NONE',  ( -4.274815082592931898E-19, -0.9999939076577903929, -0.003490651415223739937 ) ) ;
#84321=EDGE_LOOP ( 'NONE', ( #37689, #22529, #71808, #100251 ) ) ;
#84322=CARTESIAN_POINT ( 'NONE',  ( 2.699999999999946443, 12.50000000000000000, 0.2813168883297361700 ) ) ;
#84323=DIRECTION ( 'NONE',  ( -0.000000000000000000, -1.000000000000000000, -0.000000000000000000 ) ) ;
#84324=CARTESIAN_POINT ( 'NONE',  ( 11.04999999999990834, 2.500000000000000000, 1.718653347947321386 ) ) ;
#84325=CARTESIAN_POINT ( 'NONE',  ( 20.64614705758971525, -2.669560853935425637, 2.247897417627709338 ) ) ;
#84326=EDGE_CURVE ( 'NONE', #44264, #78788, #47547, .T. ) ;
#84327=CIRCLE ( 'NONE', #2851, 0.06509327318403745899 ) ;
#84328=AXIS2_PLACEMENT_3D ( 'NONE', #62713, #13583, #53534 ) ;
#84329=EDGE_CURVE ( 'NONE', #72026, #117286, #101921, .T. ) ;
#84330=CONICAL_SURFACE ( 'NONE', #27896, 0.1000000000000000472, 0.003490658503988666988 ) ;
#84331=VERTEX_POINT ( 'NONE', #73141 ) ;
#84332=EDGE_CURVE ( 'NONE', #129616, #36522, #120697, .T. ) ;
#84333=EDGE_LOOP ( 'NONE', ( #24973, #100390 ) ) ;
#84334=ORIENTED_EDGE ( 'NONE', *, *, #62308, .T. ) ;
#84335=CARTESIAN_POINT ( 'NONE',  ( 11.89999999999990443, 2.500000000000000000, 0.3464101615137736845 ) ) ;
#84336=FACE_OUTER_BOUND ( 'NONE', #12767, .T. ) ;
#84337=DIRECTION ( 'NONE',  ( 0.000000000000000000, 1.000000000000000000, 0.000000000000000000 ) ) ;
#84338=FACE_BOUND ( 'NONE', #77982, .T. ) ;
#84339=AXIS2_PLACEMENT_3D ( 'NONE', #29490, #26908, #38686 ) ;
#84340=DIRECTION ( 'NONE',  ( -0.000000000000000000, 1.000000000000000000, -0.000000000000000000 ) ) ;
#84341=DIRECTION ( 'NONE',  ( 0.000000000000000000, 1.000000000000000000, 0.000000000000000000 ) ) ;
#84342=EDGE_CURVE ( 'NONE', #119121, #36522, #13559, .T. ) ;
#84343=CARTESIAN_POINT ( 'NONE',  ( 12.69999999999990159, 2.500000000000000000, -3.983716857408426293 ) ) ;
#84344=CONICAL_SURFACE ( 'NONE', #65560, 0.1000000000000002554, 0.003490658503988666988 ) ;
#84345=AXIS2_PLACEMENT_3D ( 'NONE', #6810, #74303, #64465 ) ;
#84346=AXIS2_PLACEMENT_3D ( 'NONE', #77002, #117541, #108391 ) ;
#84348=CARTESIAN_POINT ( 'NONE',  ( 6.449999999999928235, 12.50000000000000000, 2.511473670974873507 ) ) ;
#84349=AXIS2_PLACEMENT_3D ( 'NONE', #50104, #10159, #117495 ) ;
#84350=PLANE ( 'NONE',  #55271 ) ;
#84352=CONICAL_SURFACE ( 'NONE', #17529, 0.09999999999999999167, 0.003490658503988666988 ) ;
#84353=CARTESIAN_POINT ( 'NONE',  ( -1.650000000000035660, 2.500000000000000000, 2.857883832488649301 ) ) ;
#84354=EDGE_LOOP ( 'NONE', ( #21740, #25462, #5960, #107698 ) ) ;
#84355=ORIENTED_EDGE ( 'NONE', *, *, #23064, .T. ) ;
#84356=EDGE_LOOP ( 'NONE', ( #34860, #16080, #72477, #47523 ) ) ;
#84357=ORIENTED_EDGE ( 'NONE', *, *, #97466, .F. ) ;
#84358=DIRECTION ( 'NONE',  ( 0.000000000000000000, -0.000000000000000000, 1.000000000000000000 ) ) ;
#84359=EDGE_CURVE ( 'NONE', #47322, #35537, #43706, .T. ) ;
#84360=FACE_BOUND ( 'NONE', #26051, .T. ) ;
#84362=VECTOR ( 'NONE', #97463, 1000.000000000000000 ) ;
#84363=ORIENTED_EDGE ( 'NONE', *, *, #40879, .F. ) ;
#84364=DIRECTION ( 'NONE',  ( 0.000000000000000000, 1.000000000000000000, 0.000000000000000000 ) ) ;
#84365=AXIS2_PLACEMENT_3D ( 'NONE', #71252, #50996, #39888 ) ;
#84366=CARTESIAN_POINT ( 'NONE',  ( 9.999999999999948486, 2.500000000000000000, -4.330127018922201643 ) ) ;
#84367=ORIENTED_EDGE ( 'NONE', *, *, #56962, .T. ) ;
#84368=CARTESIAN_POINT ( 'NONE',  ( -4.400000000000028777, 12.50000000000000000, -3.983716857408426293 ) ) ;
#84369=FACE_OUTER_BOUND ( 'NONE', #59534, .T. ) ;
#84370=CONICAL_SURFACE ( 'NONE', #119974, 0.1000000000000002554, 0.003490658503988666988 ) ;
#84371=AXIS2_PLACEMENT_3D ( 'NONE', #74469, #14239, #122932 ) ;
#84372=EDGE_CURVE ( 'NONE', #44029, #109510, #28771, .T. ) ;
#84373=AXIS2_PLACEMENT_3D ( 'NONE', #11601, #51548, #1769 ) ;
#84374=CONICAL_SURFACE ( 'NONE', #101100, 0.1000000000000002554, 0.003490658503988666988 ) ;
#84375=ORIENTED_EDGE ( 'NONE', *, *, #105688, .T. ) ;
#84376=CARTESIAN_POINT ( 'NONE',  ( 0.3999999999999559464, 2.500000000000000000, -4.430127018922202176 ) ) ;
#84377=CARTESIAN_POINT ( 'NONE',  ( 5.649999999999932854, 12.50000000000000000, 1.883746621131358934 ) ) ;
#84378=AXIS2_PLACEMENT_3D ( 'NONE', #51268, #111437, #42078 ) ;
#84379=EDGE_LOOP ( 'NONE', ( #14490, #31285, #71822, #129326 ) ) ;
#84380=DIRECTION ( 'NONE',  ( 0.000000000000000000, 0.000000000000000000, 1.000000000000000000 ) ) ;
#84381=CARTESIAN_POINT ( 'NONE',  ( 9.399999999999915090, 2.500000000000000000, 3.983716857408420964 ) ) ;
#84382=CARTESIAN_POINT ( 'NONE',  ( 8.349999999999923261, 2.500000000000000000, 2.165063509461097713 ) ) ;
#84383=AXIS2_PLACEMENT_3D ( 'NONE', #64147, #85080, #93616 ) ;
#84384=ORIENTED_EDGE ( 'NONE', *, *, #46646, .F. ) ;
#84385=EDGE_LOOP ( 'NONE', ( #27203, #66667, #102706, #2275 ) ) ;
#84386=EDGE_CURVE ( 'NONE', #4566, #38948, #32981, .T. ) ;
#84387=CARTESIAN_POINT ( 'NONE',  ( 9.599999999999917932, 2.500000000000000000, 0.7928203230275495672 ) ) ;
#84388=ORIENTED_EDGE ( 'NONE', *, *, #65834, .F. ) ;
#84389=CARTESIAN_POINT ( 'NONE',  ( -14.14999999999998792, 12.50000000000000000, 2.922977105672690534 ) ) ;
#84390=DIRECTION ( 'NONE',  ( -0.000000000000000000, -1.000000000000000000, -0.000000000000000000 ) ) ;
#84391=VERTEX_POINT ( 'NONE', #17915 ) ;
#84392=DIRECTION ( 'NONE',  ( 0.000000000000000000, 0.000000000000000000, -1.000000000000000000 ) ) ;
#84393=DIRECTION ( 'NONE',  ( 0.000000000000000000, 0.000000000000000000, -1.000000000000000000 ) ) ;
#84394=DIRECTION ( 'NONE',  ( 0.000000000000000000, -0.000000000000000000, 1.000000000000000000 ) ) ;
#84396=CARTESIAN_POINT ( 'NONE',  ( -3.550000000000031797, 12.50000000000000000, -6.213873640053564351 ) ) ;
#84397=CIRCLE ( 'NONE', #80210, 0.06509327318403745899 ) ;
#84398=ORIENTED_EDGE ( 'NONE', *, *, #103214, .T. ) ;
#84399=ORIENTED_EDGE ( 'NONE', *, *, #100961, .F. ) ;
#84400=DIRECTION ( 'NONE',  ( -0.000000000000000000, -1.000000000000000000, -0.000000000000000000 ) ) ;
#84401=DIRECTION ( 'NONE',  ( 0.000000000000000000, -0.000000000000000000, 1.000000000000000000 ) ) ;
#84402=DIRECTION ( 'NONE',  ( 0.000000000000000000, -0.9999939076577903929, 0.003490651415223739937 ) ) ;
#84404=VERTEX_POINT ( 'NONE', #77484 ) ;
#84405=ORIENTED_EDGE ( 'NONE', *, *, #45118, .F. ) ;
#84406=CARTESIAN_POINT ( 'NONE',  ( -3.350000000000028955, 2.500000000000000000, 2.165063509461097713 ) ) ;
#84407=CIRCLE ( 'NONE', #10936, 0.06509327318403745899 ) ;
#84408=CIRCLE ( 'NONE', #27975, 0.1000000000000000472 ) ;
#84409=CARTESIAN_POINT ( 'NONE',  ( 8.099999999999923261, 12.50000000000000000, 4.676537180435972552 ) ) ;
#84410=CIRCLE ( 'NONE', #15343, 0.06509327318403745899 ) ;
#84411=FACE_OUTER_BOUND ( 'NONE', #66600, .T. ) ;
#84412=ADVANCED_FACE ( 'NONE', ( #29053 ), #48043, .T. ) ;
#84414=CARTESIAN_POINT ( 'NONE',  ( 9.599999999999914380, 12.50000000000000000, 3.637306695894644726 ) ) ;
#84415=DIRECTION ( 'NONE',  ( -4.274815082592931898E-19, -0.9999939076577903929, -0.003490651415223739937 ) ) ;
#84416=CARTESIAN_POINT ( 'NONE',  ( -0.6000000000000383915, 2.500000000000000000, -4.576537180435977348 ) ) ;
#84418=CARTESIAN_POINT ( 'NONE',  ( 8.349999999999919709, 12.50000000000000000, -1.472243186433550122 ) ) ;
#84419=CIRCLE ( 'NONE', #17505, 0.1000000000000000472 ) ;
#84420=DIRECTION ( 'NONE',  ( -4.274815082592931898E-19, -0.9999939076577903929, -0.003490651415223739937 ) ) ;
#84421=VECTOR ( 'NONE', #112264, 1000.000000000000000 ) ;
#84422=VERTEX_POINT ( 'NONE', #129203 ) ;
#84423=VECTOR ( 'NONE', #7515, 1000.000000000000000 ) ;
#84424=PLANE ( 'NONE',  #117582 ) ;
#84425=EDGE_CURVE ( 'NONE', #3854, #8978, #45500, .T. ) ;
#84426=ORIENTED_EDGE ( 'NONE', *, *, #62293, .T. ) ;
#84427=EDGE_CURVE ( 'NONE', #103166, #79180, #83152, .T. ) ;
#84428=ORIENTED_EDGE ( 'NONE', *, *, #51081, .F. ) ;
#84429=EDGE_CURVE ( 'NONE', #94365, #118, #57862, .T. ) ;
#84430=DIRECTION ( 'NONE',  ( 0.000000000000000000, 0.000000000000000000, 1.000000000000000000 ) ) ;
#84431=DIRECTION ( 'NONE',  ( 0.000000000000000000, 0.000000000000000000, 1.000000000000000000 ) ) ;
#84432=CIRCLE ( 'NONE', #27998, 0.06509327318403745899 ) ;
#84433=ADVANCED_FACE ( 'NONE', ( #127874 ), #68454, .T. ) ;
#84434=CARTESIAN_POINT ( 'NONE',  ( 10.19999999999991047, 12.50000000000000000, 4.611443907251934426 ) ) ;
#84435=CARTESIAN_POINT ( 'NONE',  ( -12.29999999999999716, 12.50000000000000000, -4.048810130592460865 ) ) ;
#84436=LINE ( 'NONE', #3301, #100898 ) ;
#84437=AXIS2_PLACEMENT_3D ( 'NONE', #7373, #77416, #127802 ) ;
#84438=EDGE_CURVE ( 'NONE', #108779, #97111, #74730, .T. ) ;
#84439=DIRECTION ( 'NONE',  ( 0.000000000000000000, 0.000000000000000000, 1.000000000000000000 ) ) ;
#84440=VECTOR ( 'NONE', #108028, 1000.000000000000000 ) ;
#84441=CONICAL_SURFACE ( 'NONE', #15465, 0.1000000000000002554, 0.003490658503988666988 ) ;
#84442=CARTESIAN_POINT ( 'NONE',  ( 10.39999999999990976, 2.500000000000000000, -4.330127018922201643 ) ) ;
#84443=EDGE_LOOP ( 'NONE', ( #76808, #38534 ) ) ;
#84444=CARTESIAN_POINT ( 'NONE',  ( -4.600000000000024514, 12.50000000000000000, 0.6277270498435120194 ) ) ;
#84445=CIRCLE ( 'NONE', #96956, 0.09999999999999982514 ) ;
#84446=EDGE_CURVE ( 'NONE', #4103, #69263, #7815, .T. ) ;
#84447=CIRCLE ( 'NONE', #21667, 0.06509327318403745899 ) ;
#84448=DIRECTION ( 'NONE',  ( -0.000000000000000000, -1.000000000000000000, -0.000000000000000000 ) ) ;
#84449=EDGE_CURVE ( 'NONE', #1478, #47032, #28399, .T. ) ;
#84450=EDGE_LOOP ( 'NONE', ( #127148, #35645, #14992, #37596 ) ) ;
#84451=ADVANCED_FACE ( 'NONE', ( #38891 ), #20438, .T. ) ;
#84452=ORIENTED_EDGE ( 'NONE', *, *, #32359, .F. ) ;
#84453=EDGE_LOOP ( 'NONE', ( #111816, #127330, #107355, #89712 ) ) ;
#84454=ORIENTED_EDGE ( 'NONE', *, *, #126904, .F. ) ;
#84455=EDGE_CURVE ( 'NONE', #18847, #68325, #30837, .T. ) ;
#84456=DIRECTION ( 'NONE',  ( 0.000000000000000000, 1.000000000000000000, 0.000000000000000000 ) ) ;
#84457=CARTESIAN_POINT ( 'NONE',  ( -6.850000000000017408, 12.50000000000000000, -6.841600689897077814 ) ) ;
#84458=DIRECTION ( 'NONE',  ( 0.000000000000000000, 0.000000000000000000, -1.000000000000000000 ) ) ;
#84459=DIRECTION ( 'NONE',  ( 0.000000000000000000, 0.000000000000000000, -1.000000000000000000 ) ) ;
#84460=CIRCLE ( 'NONE', #107728, 0.1000000000000002554 ) ;
#84461=CARTESIAN_POINT ( 'NONE',  ( 13.54999999999989768, 2.500000000000000000, -2.411473670974877859 ) ) ;
#84462=ORIENTED_EDGE ( 'NONE', *, *, #81030, .T. ) ;
#84463=DIRECTION ( 'NONE',  ( -0.000000000000000000, -1.000000000000000000, -0.000000000000000000 ) ) ;
#84464=VECTOR ( 'NONE', #113739, 1000.000000000000000 ) ;
#84465=AXIS2_PLACEMENT_3D ( 'NONE', #59463, #37851, #126891 ) ;
#84466=DIRECTION ( 'NONE',  ( 0.000000000000000000, 0.000000000000000000, 1.000000000000000000 ) ) ;
#84467=LINE ( 'NONE', #36672, #56195 ) ;
#84468=ORIENTED_EDGE ( 'NONE', *, *, #58219, .F. ) ;
#84469=CIRCLE ( 'NONE', #11300, 0.06509327318403745899 ) ;
#84470=AXIS2_PLACEMENT_3D ( 'NONE', #54650, #42281, #52734 ) ;
#84471=AXIS2_PLACEMENT_3D ( 'NONE', #68359, #118106, #59214 ) ;
#84472=ORIENTED_EDGE ( 'NONE', *, *, #80438, .F. ) ;
#84473=AXIS2_PLACEMENT_3D ( 'NONE', #20668, #1651, #52695 ) ;
#84475=DIRECTION ( 'NONE',  ( 0.000000000000000000, 1.000000000000000000, 0.000000000000000000 ) ) ;
#84476=CARTESIAN_POINT ( 'NONE',  ( -1.250000000000035749, 12.50000000000000000, -7.188010851410854052 ) ) ;
#84478=CONICAL_SURFACE ( 'NONE', #101205, 0.1000000000000002554, 0.003490658503988666988 ) ;
#84479=AXIS2_PLACEMENT_3D ( 'NONE', #5354, #87137, #127085 ) ;
#84480=VECTOR ( 'NONE', #17620, 1000.000000000000000 ) ;
#84481=ORIENTED_EDGE ( 'NONE', *, *, #57677, .T. ) ;
#84482=CARTESIAN_POINT ( 'NONE',  ( 3.099999999999945022, 2.500000000000000000, -0.3464101615137783474 ) ) ;
#84483=DIRECTION ( 'NONE',  ( 0.000000000000000000, 0.000000000000000000, 1.000000000000000000 ) ) ;
#84484=DIRECTION ( 'NONE',  ( -4.274815082592931898E-19, -0.9999939076577903929, -0.003490651415223739937 ) ) ;
#84486=CARTESIAN_POINT ( 'NONE',  ( 4.149999999999941735, 2.500000000000000000, -7.188010851410854052 ) ) ;
#84487=EDGE_CURVE ( 'NONE', #94071, #23072, #80990, .T. ) ;
#84489=CARTESIAN_POINT ( 'NONE',  ( 105.5000000000000142, 0.000000000000000000, 0.000000000000000000 ) ) ;
#84490=EDGE_CURVE ( 'NONE', #104091, #1010, #3708, .T. ) ;
#84491=AXIS2_PLACEMENT_3D ( 'NONE', #89878, #108232, #198 ) ;
#84492=ORIENTED_EDGE ( 'NONE', *, *, #56890, .F. ) ;
#84493=ORIENTED_EDGE ( 'NONE', *, *, #59750, .F. ) ;
#84494=DIRECTION ( 'NONE',  ( -0.000000000000000000, -1.000000000000000000, -0.000000000000000000 ) ) ;
#84495=DIRECTION ( 'NONE',  ( 0.000000000000000000, 0.000000000000000000, -1.000000000000000000 ) ) ;
#84496=DIRECTION ( 'NONE',  ( 0.000000000000000000, 0.000000000000000000, -1.000000000000000000 ) ) ;
#84497=AXIS2_PLACEMENT_3D ( 'NONE', #15522, #96031, #77040 ) ;
#84498=DIRECTION ( 'NONE',  ( 0.000000000000000000, 0.000000000000000000, 1.000000000000000000 ) ) ;
#84499=ADVANCED_FACE ( 'NONE', ( #37580 ), #27732, .T. ) ;
#84501=ORIENTED_EDGE ( 'NONE', *, *, #64001, .T. ) ;
#84502=ORIENTED_EDGE ( 'NONE', *, *, #60104, .F. ) ;
#84503=DIRECTION ( 'NONE',  ( 0.000000000000000000, 0.000000000000000000, -1.000000000000000000 ) ) ;
#84504=CARTESIAN_POINT ( 'NONE',  ( 5.599999999999934808, 12.50000000000000000, -4.048810130592463530 ) ) ;
#84505=CARTESIAN_POINT ( 'NONE',  ( 7.099999999999928590, 2.500000000000000000, -4.330127018922201643 ) ) ;
#84506=CARTESIAN_POINT ( 'NONE',  ( -10.00000000000000533, 2.500000000000000000, -5.022947341949749678 ) ) ;
#84507=ORIENTED_EDGE ( 'NONE', *, *, #59895, .T. ) ;
#84508=CONICAL_SURFACE ( 'NONE', #101231, 0.09999999999999982514, 0.003490658503988666988 ) ;
#84509=DIRECTION ( 'NONE',  ( 0.000000000000000000, 0.000000000000000000, 1.000000000000000000 ) ) ;
#84510=DIRECTION ( 'NONE',  ( 0.000000000000000000, 0.000000000000000000, 1.000000000000000000 ) ) ;
#84511=ORIENTED_EDGE ( 'NONE', *, *, #45706, .F. ) ;
#84512=CARTESIAN_POINT ( 'NONE',  ( -11.24999999999996447, 12.50000000000000000, -2.230156782645135394 ) ) ;
#84513=ORIENTED_EDGE ( 'NONE', *, *, #39944, .F. ) ;
#84514=DIRECTION ( 'NONE',  ( -0.000000000000000000, 1.000000000000000000, -0.000000000000000000 ) ) ;
#84515=ORIENTED_EDGE ( 'NONE', *, *, #57497, .F. ) ;
#84516=CARTESIAN_POINT ( 'NONE',  ( -11.69999999999999574, 2.500000000000000000, 4.230127018922196669 ) ) ;
#84517=LINE ( 'NONE', #35429, #129601 ) ;
#84518=ORIENTED_EDGE ( 'NONE', *, *, #10020, .F. ) ;
#84521=DIRECTION ( 'NONE',  ( 0.000000000000000000, 0.000000000000000000, -1.000000000000000000 ) ) ;
#84522=DIRECTION ( 'NONE',  ( 0.000000000000000000, 0.000000000000000000, 1.000000000000000000 ) ) ;
#84523=CONICAL_SURFACE ( 'NONE', #44832, 0.1000000000000002554, 0.003490658503988666988 ) ;
#84524=AXIS2_PLACEMENT_3D ( 'NONE', #112043, #81292, #111370 ) ;
#84525=DIRECTION ( 'NONE',  ( 0.000000000000000000, 1.000000000000000000, 0.000000000000000000 ) ) ;
#84526=DIRECTION ( 'NONE',  ( -0.000000000000000000, -1.000000000000000000, -0.000000000000000000 ) ) ;
#84527=CARTESIAN_POINT ( 'NONE',  ( 10.84999999999990905, 2.500000000000000000, -5.802370205355749988 ) ) ;
#84528=CIRCLE ( 'NONE', #74065, 0.06509327318403745899 ) ;
#84529=DIRECTION ( 'NONE',  ( 0.000000000000000000, -0.9999939076577903929, 0.003490651415223739937 ) ) ;
#84530=AXIS2_PLACEMENT_3D ( 'NONE', #16706, #46851, #75635 ) ;
#84531=EDGE_LOOP ( 'NONE', ( #15395, #99225, #2293, #72350 ) ) ;
#84532=ORIENTED_EDGE ( 'NONE', *, *, #40689, .T. ) ;
#84533=DIRECTION ( 'NONE',  ( 0.000000000000000000, 1.000000000000000000, 0.000000000000000000 ) ) ;
#84534=CARTESIAN_POINT ( 'NONE',  ( -2.700000000000029932, 2.500000000000000000, -0.3464101615137782364 ) ) ;
#84535=LINE ( 'NONE', #102872, #72174 ) ;
#84536=ADVANCED_FACE ( 'NONE', ( #79440 ), #128554, .T. ) ;
#84537=DIRECTION ( 'NONE',  ( 0.000000000000000000, 1.000000000000000000, 0.000000000000000000 ) ) ;
#84538=ORIENTED_EDGE ( 'NONE', *, *, #105157, .T. ) ;
#84539=ORIENTED_EDGE ( 'NONE', *, *, #102634, .F. ) ;
#84540=DIRECTION ( 'NONE',  ( -0.000000000000000000, -1.000000000000000000, -0.000000000000000000 ) ) ;
#84541=ORIENTED_EDGE ( 'NONE', *, *, #1351, .F. ) ;
#84542=ADVANCED_FACE ( 'NONE', ( #49990 ), #24553, .T. ) ;
#84543=CARTESIAN_POINT ( 'NONE',  ( 8.549999999999920774, 2.500000000000000000, 6.248780366869521430 ) ) ;
#84544=DIRECTION ( 'NONE',  ( 0.000000000000000000, 0.000000000000000000, -1.000000000000000000 ) ) ;
#84545=VERTEX_POINT ( 'NONE', #15491 ) ;
#84546=CARTESIAN_POINT ( 'NONE',  ( 7.499999999999923617, 12.50000000000000000, 0.6928203230275494784 ) ) ;
#84547=DIRECTION ( 'NONE',  ( 0.000000000000000000, 0.000000000000000000, 1.000000000000000000 ) ) ;
#84548=DIRECTION ( 'NONE',  ( -0.000000000000000000, -1.000000000000000000, -0.000000000000000000 ) ) ;
#84549=VECTOR ( 'NONE', #31479, 1000.000000000000000 ) ;
#84550=CARTESIAN_POINT ( 'NONE',  ( -8.950000000000008171, 12.50000000000000000, 1.753560074763284016 ) ) ;
#84551=AXIS2_PLACEMENT_3D ( 'NONE', #4396, #113092, #23416 ) ;
#84552=DIRECTION ( 'NONE',  ( -0.000000000000000000, -1.000000000000000000, -0.000000000000000000 ) ) ;
#84553=DIRECTION ( 'NONE',  ( 0.000000000000000000, -0.9999939076577903929, 0.003490651415223739937 ) ) ;
#84554=AXIS2_PLACEMENT_3D ( 'NONE', #82844, #82181, #52715 ) ;
#84556=DIRECTION ( 'NONE',  ( 0.000000000000000000, 0.000000000000000000, 1.000000000000000000 ) ) ;
#84557=FACE_OUTER_BOUND ( 'NONE', #54982, .T. ) ;
#84558=LINE ( 'NONE', #45935, #22238 ) ;
#84559=AXIS2_PLACEMENT_3D ( 'NONE', #7127, #28079, #67987 ) ;
#84560=EDGE_LOOP ( 'NONE', ( #85289, #70251, #122634, #7343 ) ) ;
#84561=VERTEX_POINT ( 'NONE', #81995 ) ;
#84562=ORIENTED_EDGE ( 'NONE', *, *, #91212, .T. ) ;
#84563=DIRECTION ( 'NONE',  ( -0.000000000000000000, 1.000000000000000000, -0.000000000000000000 ) ) ;
#84564=ORIENTED_EDGE ( 'NONE', *, *, #71309, .F. ) ;
#84565=DIRECTION ( 'NONE',  ( -0.000000000000000000, 1.000000000000000000, -0.000000000000000000 ) ) ;
#84566=VERTEX_POINT ( 'NONE', #62376 ) ;
#84567=EDGE_LOOP ( 'NONE', ( #26778, #18803, #14598, #47508 ) ) ;
#84568=VERTEX_POINT ( 'NONE', #61069 ) ;
#84569=CARTESIAN_POINT ( 'NONE',  ( -5.600000000000020073, 2.500000000000000000, 3.983716857408420964 ) ) ;
#84570=CONICAL_SURFACE ( 'NONE', #103450, 0.09999999999999999167, 0.003490658503988666988 ) ;
#84571=DIRECTION ( 'NONE',  ( 0.000000000000000000, 0.000000000000000000, 1.000000000000000000 ) ) ;
#84572=EDGE_CURVE ( 'NONE', #128871, #55439, #58014, .T. ) ;
#84573=CARTESIAN_POINT ( 'NONE',  ( 12.89999999999989733, 12.50000000000000000, -2.385244779468109755E-15 ) ) ;
#84574=CARTESIAN_POINT ( 'NONE',  ( -8.350000000000013856, 2.500000000000000000, -2.065063509461102065 ) ) ;
#84575=AXIS2_PLACEMENT_3D ( 'NONE', #77046, #58062, #97965 ) ;
#84576=CARTESIAN_POINT ( 'NONE',  ( -6.900000000000019007, 2.500000000000000000, -0.2464101615137783419 ) ) ;
#84577=ORIENTED_EDGE ( 'NONE', *, *, #38627, .T. ) ;
#84578=DIRECTION ( 'NONE',  ( 0.000000000000000000, 0.000000000000000000, -1.000000000000000000 ) ) ;
#84579=ORIENTED_EDGE ( 'NONE', *, *, #104284, .F. ) ;
#84580=EDGE_CURVE ( 'NONE', #35226, #97598, #21142, .T. ) ;
#84581=ORIENTED_EDGE ( 'NONE', *, *, #80139, .T. ) ;
#84582=EDGE_LOOP ( 'NONE', ( #104894, #69905 ) ) ;
#84583=DIRECTION ( 'NONE',  ( 0.000000000000000000, 1.000000000000000000, 0.000000000000000000 ) ) ;
#84585=EDGE_CURVE ( 'NONE', #47459, #37524, #120637, .T. ) ;
#84586=ORIENTED_EDGE ( 'NONE', *, *, #114404, .T. ) ;
#84587=EDGE_CURVE ( 'NONE', #4707, #85507, #16209, .T. ) ;
#84588=ORIENTED_EDGE ( 'NONE', *, *, #36327, .T. ) ;
#84589=EDGE_CURVE ( 'NONE', #93106, #111188, #51751, .T. ) ;
#84590=EDGE_LOOP ( 'NONE', ( #83256, #112251, #118988, #107399 ) ) ;
#84591=EDGE_CURVE ( 'NONE', #74727, #103978, #12020, .T. ) ;
#84592=VECTOR ( 'NONE', #44691, 1000.000000000000000 ) ;
#84593=DIRECTION ( 'NONE',  ( -0.000000000000000000, 1.000000000000000000, -0.000000000000000000 ) ) ;
#84594=CARTESIAN_POINT ( 'NONE',  ( -13.74999999999995381, 12.50000000000000000, 2.099970236277064028 ) ) ;
#84595=CARTESIAN_POINT ( 'NONE',  ( 2.699999999999947331, 12.50000000000000000, -0.2813168883297409439 ) ) ;
#84596=DIRECTION ( 'NONE',  ( 0.000000000000000000, 0.000000000000000000, 1.000000000000000000 ) ) ;
#84597=EDGE_CURVE ( 'NONE', #72456, #40560, #66491, .T. ) ;
#84598=CARTESIAN_POINT ( 'NONE',  ( 11.24999999999991118, 12.50000000000000000, 5.802370205355744659 ) ) ;
#84599=EDGE_LOOP ( 'NONE', ( #82023, #53838, #67982, #61967 ) ) ;
#84600=ADVANCED_FACE ( 'NONE', ( #92458 ), #81091, .T. ) ;
#84601=DIRECTION ( 'NONE',  ( 0.000000000000000000, 1.000000000000000000, 0.000000000000000000 ) ) ;
#84602=AXIS2_PLACEMENT_3D ( 'NONE', #17383, #97252, #47521 ) ;
#84603=AXIS2_PLACEMENT_3D ( 'NONE', #17528, #86916, #124921 ) ;
#84604=ADVANCED_FACE ( 'NONE', ( #864 ), #56024, .T. ) ;
#84605=ORIENTED_EDGE ( 'NONE', *, *, #17149, .F. ) ;
#84606=DIRECTION ( 'NONE',  ( 0.000000000000000000, 0.000000000000000000, -1.000000000000000000 ) ) ;
#84607=ADVANCED_FACE ( 'NONE', ( #70252 ), #89487, .T. ) ;
#84608=ORIENTED_EDGE ( 'NONE', *, *, #9213, .T. ) ;
#84609=ORIENTED_EDGE ( 'NONE', *, *, #61176, .F. ) ;
#84610=VERTEX_POINT ( 'NONE', #111447 ) ;
#84611=EDGE_CURVE ( 'NONE', #41152, #10139, #16304, .T. ) ;
#84612=CARTESIAN_POINT ( 'NONE',  ( 12.09999999999990195, 12.50000000000000000, -0.6928203230275541413 ) ) ;
#84613=DIRECTION ( 'NONE',  ( 0.000000000000000000, 1.000000000000000000, 0.000000000000000000 ) ) ;
#84614=CONICAL_SURFACE ( 'NONE', #40717, 0.1000000000000000472, 0.003490658503988666988 ) ;
#84615=CARTESIAN_POINT ( 'NONE',  ( 6.249999999999930722, 2.500000000000000000, 7.188010851410848723 ) ) ;
#84616=CIRCLE ( 'NONE', #36512, 0.1000000000000000472 ) ;
#84617=ORIENTED_EDGE ( 'NONE', *, *, #91078, .T. ) ;
#84618=CARTESIAN_POINT ( 'NONE',  ( 5.199999999999933564, 2.500000000000000000, 4.083716857408420609 ) ) ;
#84619=ORIENTED_EDGE ( 'NONE', *, *, #53512, .T. ) ;
#84620=DIRECTION ( 'NONE',  ( 0.000000000000000000, 1.000000000000000000, 0.000000000000000000 ) ) ;
#84621=CARTESIAN_POINT ( 'NONE',  ( -1.850000000000033396, 2.500000000000000000, -1.718653347947325827 ) ) ;
#84622=CARTESIAN_POINT ( 'NONE',  ( 6.649999999999927525, 2.500000000000000000, 2.065063509461097624 ) ) ;
#84623=CARTESIAN_POINT ( 'NONE',  ( -12.49999999999995737, 12.50000000000000000, 4.265033745738159077 ) ) ;
#84624=CARTESIAN_POINT ( 'NONE',  ( -10.45000000000000107, 12.50000000000000000, 2.099970236277060032 ) ) ;
#84625=ORIENTED_EDGE ( 'NONE', *, *, #118549, .T. ) ;
#84626=AXIS2_PLACEMENT_3D ( 'NONE', #74369, #11081, #90280 ) ;
#84627=AXIS2_PLACEMENT_3D ( 'NONE', #48815, #69073, #28520 ) ;
#84628=ORIENTED_EDGE ( 'NONE', *, *, #11719, .T. ) ;
#84629=CIRCLE ( 'NONE', #101062, 0.1000000000000002554 ) ;
#84630=EDGE_LOOP ( 'NONE', ( #128047, #23955, #73229, #109542 ) ) ;
#84631=VECTOR ( 'NONE', #19294, 1000.000000000000000 ) ;
#84633=DIRECTION ( 'NONE',  ( 0.000000000000000000, 0.000000000000000000, 1.000000000000000000 ) ) ;
#84635=DIRECTION ( 'NONE',  ( -4.274815082592931898E-19, -0.9999939076577903929, -0.003490651415223739937 ) ) ;
#84636=CARTESIAN_POINT ( 'NONE',  ( 7.699999999999923794, 2.500000000000000000, 4.676537180435972552 ) ) ;
#84637=LINE ( 'NONE', #122632, #4209 ) ;
#84638=CARTESIAN_POINT ( 'NONE',  ( 8.099999999999923261, 2.500000000000000000, 3.983716857408420076 ) ) ;
#84639=EDGE_LOOP ( 'NONE', ( #82599, #100465, #12677, #125303 ) ) ;
#84640=EDGE_CURVE ( 'NONE', #97955, #56748, #43385, .T. ) ;
#84641=CIRCLE ( 'NONE', #49156, 0.09999999999999982514 ) ;
#84642=DIRECTION ( 'NONE',  ( 0.000000000000000000, 0.000000000000000000, 1.000000000000000000 ) ) ;
#84643=CARTESIAN_POINT ( 'NONE',  ( -0.2000000000000399791, 2.500000000000000000, -4.676537180435977881 ) ) ;
#84644=CONICAL_SURFACE ( 'NONE', #19802, 0.1000000000000002554, 0.003490658503988666988 ) ;
#84645=ADVANCED_FACE ( 'NONE', ( #32928 ), #124993, .T. ) ;
#84646=ORIENTED_EDGE ( 'NONE', *, *, #14795, .T. ) ;
#84647=CIRCLE ( 'NONE', #47003, 0.06509327318403741736 ) ;
#84648=DIRECTION ( 'NONE',  ( 0.000000000000000000, 0.000000000000000000, 1.000000000000000000 ) ) ;
#84649=AXIS2_PLACEMENT_3D ( 'NONE', #115640, #56706, #114360 ) ;
#84650=EDGE_LOOP ( 'NONE', ( #107826, #23382, #21680, #25391 ) ) ;
#84651=AXIS2_PLACEMENT_3D ( 'NONE', #8746, #48704, #38907 ) ;
#84652=DIRECTION ( 'NONE',  ( 0.000000000000000000, -0.000000000000000000, 1.000000000000000000 ) ) ;
#84653=CIRCLE ( 'NONE', #124376, 0.1000000000000000472 ) ;
#84654=VERTEX_POINT ( 'NONE', #3437 ) ;
#84655=DIRECTION ( 'NONE',  ( 0.000000000000000000, 0.000000000000000000, 1.000000000000000000 ) ) ;
#84656=CARTESIAN_POINT ( 'NONE',  ( -2.050000000000033129, 12.50000000000000000, 2.165063509461097713 ) ) ;
#84657=CARTESIAN_POINT ( 'NONE',  ( -7.900000000000011013, 2.500000000000000000, 4.922947341949748257 ) ) ;
#84658=EDGE_LOOP ( 'NONE', ( #64739, #61638, #56801, #77453 ) ) ;
#84659=AXIS2_PLACEMENT_3D ( 'NONE', #88110, #77038, #87482 ) ;
#84660=AXIS2_PLACEMENT_3D ( 'NONE', #101770, #23193, #63125 ) ;
#84662=DIRECTION ( 'NONE',  ( 0.000000000000000000, 0.000000000000000000, 1.000000000000000000 ) ) ;
#84663=ORIENTED_EDGE ( 'NONE', *, *, #4075, .T. ) ;
#84664=CARTESIAN_POINT ( 'NONE',  ( 5.649999999999936406, 2.500000000000000000, -6.148780366869526226 ) ) ;
#84665=ORIENTED_EDGE ( 'NONE', *, *, #118114, .T. ) ;
#84666=ORIENTED_EDGE ( 'NONE', *, *, #39437, .T. ) ;
#84667=CARTESIAN_POINT ( 'NONE',  ( 1.849999999999948130, 12.50000000000000000, 6.213873640053558134 ) ) ;
#84668=DIRECTION ( 'NONE',  ( 0.000000000000000000, 0.000000000000000000, -1.000000000000000000 ) ) ;
#84669=VERTEX_POINT ( 'NONE', #82660 ) ;
#84670=DIRECTION ( 'NONE',  ( 0.000000000000000000, -0.000000000000000000, 1.000000000000000000 ) ) ;
#84671=DIRECTION ( 'NONE',  ( 0.000000000000000000, 1.000000000000000000, 0.000000000000000000 ) ) ;
#84672=AXIS2_PLACEMENT_3D ( 'NONE', #71487, #111401, #49306 ) ;
#84673=VERTEX_POINT ( 'NONE', #112760 ) ;
#84674=DIRECTION ( 'NONE',  ( 0.000000000000000000, 0.000000000000000000, 1.000000000000000000 ) ) ;
#84675=ADVANCED_FACE ( 'NONE', ( #20514 ), #37273, .T. ) ;
#84676=FACE_OUTER_BOUND ( 'NONE', #93604, .T. ) ;
#84678=CARTESIAN_POINT ( 'NONE',  ( 17.49862860983166257, -2.500000000000000000, -4.081131818001380474 ) ) ;
#84679=FACE_OUTER_BOUND ( 'NONE', #34519, .T. ) ;
#84680=PLANE ( 'NONE',  #5439 ) ;
#84681=DIRECTION ( 'NONE',  ( 0.000000000000000000, 0.000000000000000000, 1.000000000000000000 ) ) ;
#84682=CIRCLE ( 'NONE', #82554, 0.06509327318403745899 ) ;
#84683=CONICAL_SURFACE ( 'NONE', #24149, 0.09999999999999982514, 0.003490658503988666988 ) ;
#84684=ORIENTED_EDGE ( 'NONE', *, *, #116327, .F. ) ;
#84685=VERTEX_POINT ( 'NONE', #10653 ) ;
#84686=ORIENTED_EDGE ( 'NONE', *, *, #24187, .T. ) ;
#84687=VERTEX_POINT ( 'NONE', #50599 ) ;
#84688=CARTESIAN_POINT ( 'NONE',  ( 21.23528140090950700, 2.699413673072311948, 2.293764360948889802 ) ) ;
#84689=DIRECTION ( 'NONE',  ( 0.000000000000000000, 0.000000000000000000, 1.000000000000000000 ) ) ;
#84690=ADVANCED_FACE ( 'NONE', ( #31621 ), #23085, .T. ) ;
#84691=DIRECTION ( 'NONE',  ( 0.000000000000000000, 0.000000000000000000, 1.000000000000000000 ) ) ;
#84692=ORIENTED_EDGE ( 'NONE', *, *, #6701, .F. ) ;
#84693=FACE_BOUND ( 'NONE', #55912, .T. ) ;
#84694=ADVANCED_FACE ( 'NONE', ( #105514 ), #110407, .T. ) ;
#84695=CARTESIAN_POINT ( 'NONE',  ( 12.49999999999990585, 12.50000000000000000, -5.022947341949754119 ) ) ;
#84696=CARTESIAN_POINT ( 'NONE',  ( -7.950000000000009059, 12.50000000000000000, 6.495190528383297135 ) ) ;
#84697=AXIS2_PLACEMENT_3D ( 'NONE', #49896, #61641, #89798 ) ;
#84698=CARTESIAN_POINT ( 'NONE',  ( -2.900000000000030109, 2.500000000000000000, 0.7928203230275495672 ) ) ;
#84699=DIRECTION ( 'NONE',  ( -4.274815082592931898E-19, -0.9999939076577903929, -0.003490651415223739937 ) ) ;
#84700=CONICAL_SURFACE ( 'NONE', #24072, 0.1000000000000000472, 0.003490658503988666988 ) ;
#84701=FACE_OUTER_BOUND ( 'NONE', #67567, .T. ) ;
#84702=CARTESIAN_POINT ( 'NONE',  ( -10.40000000000000213, 2.500000000000000000, 0.6928203230275494784 ) ) ;
#84703=DIRECTION ( 'NONE',  ( 0.000000000000000000, 1.000000000000000000, 0.000000000000000000 ) ) ;
#84704=CARTESIAN_POINT ( 'NONE',  ( 3.149999999999946176, 2.500000000000000000, -6.248780366869526759 ) ) ;
#84705=ADVANCED_FACE ( 'NONE', ( #34855 ), #1647, .T. ) ;
#84706=DIRECTION ( 'NONE',  ( 0.000000000000000000, 0.000000000000000000, -1.000000000000000000 ) ) ;
#84707=CARTESIAN_POINT ( 'NONE',  ( -6.050000000000022027, 2.500000000000000000, -1.718653347947326049 ) ) ;
#84708=AXIS2_PLACEMENT_3D ( 'NONE', #128658, #118157, #120736 ) ;
#84709=VERTEX_POINT ( 'NONE', #15824 ) ;
#84710=ORIENTED_EDGE ( 'NONE', *, *, #121225, .T. ) ;
#84711=VECTOR ( 'NONE', #117345, 1000.000000000000000 ) ;
#84712=EDGE_LOOP ( 'NONE', ( #10952, #45630, #120825, #69930 ) ) ;
#84714=DIRECTION ( 'NONE',  ( 0.000000000000000000, 1.000000000000000000, 0.000000000000000000 ) ) ;
#84715=ORIENTED_EDGE ( 'NONE', *, *, #11944, .T. ) ;
#84716=DIRECTION ( 'NONE',  ( 0.000000000000000000, 0.000000000000000000, 1.000000000000000000 ) ) ;
#84718=EDGE_LOOP ( 'NONE', ( #122047, #101291, #10109, #117310 ) ) ;
#84719=AXIS2_PLACEMENT_3D ( 'NONE', #103243, #43702, #113049 ) ;
#84720=LINE ( 'NONE', #35634, #78981 ) ;
#84721=DIRECTION ( 'NONE',  ( 0.000000000000000000, 0.000000000000000000, 1.000000000000000000 ) ) ;
#84722=CARTESIAN_POINT ( 'NONE',  ( -8.100000000000013856, 12.50000000000000000, -0.4115034346978156399 ) ) ;
#84723=CARTESIAN_POINT ( 'NONE',  ( 0.8499999999999536815, 12.50000000000000000, 5.867463478539781896 ) ) ;
#84724=ORIENTED_EDGE ( 'NONE', *, *, #64887, .F. ) ;
#84725=ORIENTED_EDGE ( 'NONE', *, *, #25035, .T. ) ;
#84726=EDGE_CURVE ( 'NONE', #3657, #44118, #87324, .T. ) ;
#84727=AXIS2_PLACEMENT_3D ( 'NONE', #89377, #120124, #30472 ) ;
#84728=EDGE_LOOP ( 'NONE', ( #63006, #44211 ) ) ;
#84729=DIRECTION ( 'NONE',  ( 0.000000000000000000, 1.000000000000000000, 0.000000000000000000 ) ) ;
#84730=ORIENTED_EDGE ( 'NONE', *, *, #53365, .T. ) ;
#84731=CIRCLE ( 'NONE', #76330, 0.1000000000000002554 ) ;
#84732=CIRCLE ( 'NONE', #76331, 0.1000000000000002554 ) ;
#84733=CARTESIAN_POINT ( 'NONE',  ( 3.749999999999976907, 2.500000000000000000, 2.165063509461097713 ) ) ;
#84734=ORIENTED_EDGE ( 'NONE', *, *, #14231, .T. ) ;
#84735=EDGE_CURVE ( 'NONE', #120064, #6156, #4074, .T. ) ;
#84736=VERTEX_POINT ( 'NONE', #5360 ) ;
#84737=EDGE_CURVE ( 'NONE', #20333, #98360, #85850, .T. ) ;
#84738=CARTESIAN_POINT ( 'NONE',  ( -10.60000000000000320, 2.500000000000000000, -4.576537180435972907 ) ) ;
#84739=AXIS2_PLACEMENT_3D ( 'NONE', #47903, #87798, #127109 ) ;
#84740=CIRCLE ( 'NONE', #109790, 2.000000000000000000 ) ;
#84741=CONICAL_SURFACE ( 'NONE', #117895, 0.09999999999999982514, 0.003490658503988666988 ) ;
#84742=DIRECTION ( 'NONE',  ( -0.000000000000000000, -1.000000000000000000, -0.000000000000000000 ) ) ;
#84743=CARTESIAN_POINT ( 'NONE',  ( -1.900000000000035438, 2.500000000000000000, 3.983716857408420076 ) ) ;
#84744=CARTESIAN_POINT ( 'NONE',  ( -8.749999999999975131, 2.500000000000000000, 2.165063509461097713 ) ) ;
#84745=EDGE_CURVE ( 'NONE', #61621, #19851, #45312, .T. ) ;
#84746=AXIS2_PLACEMENT_3D ( 'NONE', #80938, #59384, #81569 ) ;
#84747=EDGE_CURVE ( 'NONE', #47889, #22314, #74821, .T. ) ;
#84748=FACE_OUTER_BOUND ( 'NONE', #1699, .T. ) ;
#84749=EDGE_CURVE ( 'NONE', #39552, #64505, #60268, .T. ) ;
#84750=EDGE_CURVE ( 'NONE', #44501, #105738, #103586, .T. ) ;
#84751=ORIENTED_EDGE ( 'NONE', *, *, #3046, .F. ) ;
#84752=CARTESIAN_POINT ( 'NONE',  ( -11.44999999999999751, 12.50000000000000000, 6.906693963081109722 ) ) ;
#84753=AXIS2_PLACEMENT_3D ( 'NONE', #95243, #65110, #92657 ) ;
#84754=AXIS2_PLACEMENT_3D ( 'NONE', #128526, #29018, #38859 ) ;
#84755=ORIENTED_EDGE ( 'NONE', *, *, #118049, .F. ) ;
#84756=DIRECTION ( 'NONE',  ( 0.000000000000000000, -0.000000000000000000, 1.000000000000000000 ) ) ;
#84757=AXIS2_PLACEMENT_3D ( 'NONE', #89238, #81988, #60449 ) ;
#84758=EDGE_CURVE ( 'NONE', #117920, #53276, #99954, .T. ) ;
#84759=VERTEX_POINT ( 'NONE', #46576 ) ;
#84760=DIRECTION ( 'NONE',  ( 0.000000000000000000, 0.000000000000000000, 1.000000000000000000 ) ) ;
#84761=CARTESIAN_POINT ( 'NONE',  ( -0.8500000000000395017, 2.500000000000000000, 2.265063509461097357 ) ) ;
#84762=AXIS2_PLACEMENT_3D ( 'NONE', #103459, #15696, #13770 ) ;
#84763=DIRECTION ( 'NONE',  ( 0.000000000000000000, -0.000000000000000000, 1.000000000000000000 ) ) ;
#84764=DIRECTION ( 'NONE',  ( -0.000000000000000000, 1.000000000000000000, -0.000000000000000000 ) ) ;
#84765=ORIENTED_EDGE ( 'NONE', *, *, #107531, .T. ) ;
#84766=EDGE_CURVE ( 'NONE', #91186, #122791, #76969, .T. ) ;
#84767=PRESENTATION_STYLE_ASSIGNMENT (( #83490 ) ) ;
#84768=CARTESIAN_POINT ( 'NONE',  ( -12.89999999999999147, 12.50000000000000000, -5.022947341949751454 ) ) ;
#84769=ORIENTED_EDGE ( 'NONE', *, *, #68252, .T. ) ;
#84770=EDGE_LOOP ( 'NONE', ( #75215, #96954 ) ) ;
#84771=ORIENTED_EDGE ( 'NONE', *, *, #97027, .F. ) ;
#84772=CARTESIAN_POINT ( 'NONE',  ( -4.800000000000022915, 2.500000000000000000, 3.983716857408420076 ) ) ;
#84773=CARTESIAN_POINT ( 'NONE',  ( 3.949999999999941558, 2.500000000000000000, -6.148780366869526226 ) ) ;
#84775=AXIS2_PLACEMENT_3D ( 'NONE', #125106, #55078, #64880 ) ;
#84776=CARTESIAN_POINT ( 'NONE',  ( 4.149999999999936406, 2.500000000000000000, 6.495190528383297135 ) ) ;
#84777=DIRECTION ( 'NONE',  ( 0.000000000000000000, 1.000000000000000000, 0.000000000000000000 ) ) ;
#84778=FACE_OUTER_BOUND ( 'NONE', #110208, .T. ) ;
#84779=VECTOR ( 'NONE', #108844, 1000.000000000000000 ) ;
#84780=VERTEX_POINT ( 'NONE', #45956 ) ;
#84781=CIRCLE ( 'NONE', #38843, 0.06509327318403745899 ) ;
#84782=CARTESIAN_POINT ( 'NONE',  ( -1.250000000000035749, 2.500000000000000000, -7.088010851410853519 ) ) ;
#84783=ORIENTED_EDGE ( 'NONE', *, *, #97147, .T. ) ;
#84784=CARTESIAN_POINT ( 'NONE',  ( 6.449999999999930012, 2.500000000000000000, 6.741600689897071952 ) ) ;
#84785=CARTESIAN_POINT ( 'NONE',  ( 13.54999999999989946, 2.500000000000000000, 2.411473670974873862 ) ) ;
#84786=PLANE ( 'NONE',  #110732 ) ;
#84788=CONICAL_SURFACE ( 'NONE', #82752, 0.1000000000000000472, 0.003490658503988666988 ) ;
#84789=EDGE_CURVE ( 'NONE', #119412, #71724, #124516, .T. ) ;
#84790=DIRECTION ( 'NONE',  ( 0.000000000000000000, -0.9999939076577903929, 0.003490651415223739937 ) ) ;
#84791=DIRECTION ( 'NONE',  ( -0.000000000000000000, -1.000000000000000000, -0.000000000000000000 ) ) ;
#84792=ORIENTED_EDGE ( 'NONE', *, *, #17607, .T. ) ;
#84793=DIRECTION ( 'NONE',  ( 0.000000000000000000, 0.000000000000000000, 1.000000000000000000 ) ) ;
#84794=ADVANCED_FACE ( 'NONE', ( #115969 ), #68547, .T. ) ;
#84795=CIRCLE ( 'NONE', #122887, 0.1000000000000002554 ) ;
#84796=EDGE_LOOP ( 'NONE', ( #10988, #42256, #114260, #14062 ) ) ;
#84797=ORIENTED_EDGE ( 'NONE', *, *, #38679, .F. ) ;
#84798=DIRECTION ( 'NONE',  ( 0.000000000000000000, 0.000000000000000000, 1.000000000000000000 ) ) ;
#84799=ORIENTED_EDGE ( 'NONE', *, *, #97921, .F. ) ;
#84800=CARTESIAN_POINT ( 'NONE',  ( -5.200000000000020606, 2.500000000000000000, -0.2464101615137782308 ) ) ;
#84801=CARTESIAN_POINT ( 'NONE',  ( 10.19999999999991047, 2.500000000000000000, 4.676537180435972552 ) ) ;
#84802=CARTESIAN_POINT ( 'NONE',  ( 7.699999999999923794, 12.50000000000000000, -4.048810130592463530 ) ) ;
#84803=ORIENTED_EDGE ( 'NONE', *, *, #123477, .T. ) ;
#84804=FACE_BOUND ( 'NONE', #29319, .T. ) ;
#84805=DIRECTION ( 'NONE',  ( 0.000000000000000000, 1.000000000000000000, 0.000000000000000000 ) ) ;
#84806=LINE ( 'NONE', #16050, #6069 ) ;
#84807=ORIENTED_EDGE ( 'NONE', *, *, #21504, .T. ) ;
#84808=DIRECTION ( 'NONE',  ( 0.000000000000000000, 0.000000000000000000, 1.000000000000000000 ) ) ;
#84809=CARTESIAN_POINT ( 'NONE',  ( -12.94999999999999218, 12.50000000000000000, -2.230156782645137170 ) ) ;
#84810=EDGE_LOOP ( 'NONE', ( #12554, #114307 ) ) ;
#84811=VECTOR ( 'NONE', #101632, 1000.000000000000000 ) ;
#84812=VERTEX_POINT ( 'NONE', #63662 ) ;
#84813=AXIS2_PLACEMENT_3D ( 'NONE', #106200, #74806, #125192 ) ;
#84814=ORIENTED_EDGE ( 'NONE', *, *, #93890, .F. ) ;
#84815=CARTESIAN_POINT ( 'NONE',  ( 4.999999999999969802, 12.50000000000000000, 4.395220292106234439 ) ) ;
#84816=CARTESIAN_POINT ( 'NONE',  ( -12.04999999999999716, 2.500000000000000000, -2.065063509461098068 ) ) ;
#84817=CARTESIAN_POINT ( 'NONE',  ( -13.34999999999999076, 2.500000000000000000, -2.857883832488651521 ) ) ;
#84818=APPLICATION_CONTEXT ( 'automotive_design' ) ;
#84819=FACE_BOUND ( 'NONE', #2771, .T. ) ;
#84820=EDGE_LOOP ( 'NONE', ( #31067, #95050 ) ) ;
#84822=PLANE ( 'NONE',  #126308 ) ;
#84823=CARTESIAN_POINT ( 'NONE',  ( 2.499999999999947153, 12.50000000000000000, 3.702399969078682407 ) ) ;
#84824=ADVANCED_FACE ( 'NONE', ( #16461 ), #56395, .T. ) ;
#84825=DIRECTION ( 'NONE',  ( 0.000000000000000000, 0.000000000000000000, 1.000000000000000000 ) ) ;
#84826=B_SPLINE_CURVE_WITH_KNOTS ( 'NONE', 3,
 ( #71939, #123586, #61479, #101391, #1249, #11707 ),
 .UNSPECIFIED., .F., .F.,
 ( 4, 2, 4 ),
 ( 0.000000000000000000, 0.5000000000000000000, 1.000000000000000000 ),
 .UNSPECIFIED. ) ;
#84827=DIRECTION ( 'NONE',  ( 0.000000000000000000, -0.9999939076577903929, 0.003490651415223739937 ) ) ;
#84830=CARTESIAN_POINT ( 'NONE',  ( -14.14999999999998614, 2.500000000000000000, 1.472243186433549456 ) ) ;
#84831=CONICAL_SURFACE ( 'NONE', #109893, 0.09999999999999982514, 0.003490658503988666988 ) ;
#84832=AXIS2_PLACEMENT_3D ( 'NONE', #49153, #2586, #60880 ) ;
#84833=EDGE_CURVE ( 'NONE', #52780, #56136, #47634, .T. ) ;
#84834=DIRECTION ( 'NONE',  ( 0.000000000000000000, -0.000000000000000000, 1.000000000000000000 ) ) ;
#84835=AXIS2_PLACEMENT_3D ( 'NONE', #7284, #37420, #77328 ) ;
#84836=EDGE_LOOP ( 'NONE', ( #128151, #56921 ) ) ;
#84837=VERTEX_POINT ( 'NONE', #113386 ) ;
#84838=VERTEX_POINT ( 'NONE', #25013 ) ;
#84839=ORIENTED_EDGE ( 'NONE', *, *, #99982, .T. ) ;
#84840=CONICAL_SURFACE ( 'NONE', #99529, 0.1000000000000002554, 0.003490658503988666988 ) ;
#84841=ORIENTED_EDGE ( 'NONE', *, *, #66063, .F. ) ;
#84843=EDGE_CURVE ( 'NONE', #116415, #101569, #14160, .T. ) ;
#84844=CARTESIAN_POINT ( 'NONE',  ( -7.100000000000014744, 12.50000000000000000, 4.330127018922196314 ) ) ;
#84845=ORIENTED_EDGE ( 'NONE', *, *, #83241, .F. ) ;
#84846=FACE_BOUND ( 'NONE', #25904, .T. ) ;
#84847=EDGE_CURVE ( 'NONE', #93338, #49329, #14529, .T. ) ;
#84848=DIRECTION ( 'NONE',  ( 0.000000000000000000, 0.000000000000000000, 1.000000000000000000 ) ) ;
#84849=ADVANCED_FACE ( 'NONE', ( #44659 ), #127092, .T. ) ;
#84850=DIRECTION ( 'NONE',  ( 0.000000000000000000, -0.9999939076577903929, 0.003490651415223739937 ) ) ;
#84851=EDGE_LOOP ( 'NONE', ( #69147, #125885, #98670, #30855 ) ) ;
#84852=DIRECTION ( 'NONE',  ( 0.000000000000000000, 0.000000000000000000, -1.000000000000000000 ) ) ;
#84853=DIRECTION ( 'NONE',  ( -0.000000000000000000, -1.000000000000000000, -0.000000000000000000 ) ) ;
#84854=EDGE_CURVE ( 'NONE', #125708, #35689, #91546, .T. ) ;
#84855=DIRECTION ( 'NONE',  ( 0.000000000000000000, 1.000000000000000000, 0.000000000000000000 ) ) ;
#84856=CONICAL_SURFACE ( 'NONE', #59856, 0.09999999999999982514, 0.003490658503988666988 ) ;
#84857=ORIENTED_EDGE ( 'NONE', *, *, #54871, .T. ) ;
#84858=CARTESIAN_POINT ( 'NONE',  ( 6.649999999999930189, 12.50000000000000000, 7.253104124594885960 ) ) ;
#84859=ORIENTED_EDGE ( 'NONE', *, *, #10262, .T. ) ;
#84860=ORIENTED_EDGE ( 'NONE', *, *, #16992, .F. ) ;
#84861=ORIENTED_EDGE ( 'NONE', *, *, #52775, .F. ) ;
#84862=CARTESIAN_POINT ( 'NONE',  ( 9.999999999999948486, 2.500000000000000000, -4.430127018922202176 ) ) ;
#84863=DIRECTION ( 'NONE',  ( -0.000000000000000000, -1.000000000000000000, -0.000000000000000000 ) ) ;
#84864=CIRCLE ( 'NONE', #9568, 0.06509327318403741736 ) ;
#84865=DIRECTION ( 'NONE',  ( 0.000000000000000000, 0.000000000000000000, 1.000000000000000000 ) ) ;
#84866=EDGE_LOOP ( 'NONE', ( #32381, #67416, #104239, #21688 ) ) ;
#84867=CARTESIAN_POINT ( 'NONE',  ( 10.28037028451818458, 2.500000000000381029, -9.136909653096239481 ) ) ;
#84868=VECTOR ( 'NONE', #42030, 1000.000000000000000 ) ;
#84869=AXIS2_PLACEMENT_3D ( 'NONE', #64395, #53939, #94488 ) ;
#84870=DIRECTION ( 'NONE',  ( 0.000000000000000000, 1.000000000000000000, 0.000000000000000000 ) ) ;
#84871=AXIS2_PLACEMENT_3D ( 'NONE', #20933, #40607, #30127 ) ;
#84872=DIRECTION ( 'NONE',  ( -0.000000000000000000, 1.000000000000000000, -0.000000000000000000 ) ) ;
#84875=CARTESIAN_POINT ( 'NONE',  ( 8.349999999999919709, 12.50000000000000000, -1.472243186433550122 ) ) ;
#84876=VERTEX_POINT ( 'NONE', #59665 ) ;
#84877=DIRECTION ( 'NONE',  ( 0.000000000000000000, 0.000000000000000000, 1.000000000000000000 ) ) ;
#84878=CIRCLE ( 'NONE', #120484, 0.06509327318403745899 ) ;
#84879=ORIENTED_EDGE ( 'NONE', *, *, #111624, .F. ) ;
#84880=AXIS2_PLACEMENT_3D ( 'NONE', #56852, #5183, #106613 ) ;
#84881=VECTOR ( 'NONE', #22429, 1000.000000000000000 ) ;
#84882=ORIENTED_EDGE ( 'NONE', *, *, #96371, .F. ) ;
#84883=LINE ( 'NONE', #82320, #78488 ) ;
#84885=CARTESIAN_POINT ( 'NONE',  ( 3.299999999999944755, 2.500000000000000000, -4.330127018922201643 ) ) ;
#84886=DIRECTION ( 'NONE',  ( 0.000000000000000000, 0.000000000000000000, -1.000000000000000000 ) ) ;
#84887=CARTESIAN_POINT ( 'NONE',  ( -10.40000000000000213, 2.500000000000000000, 5.022947341949748790 ) ) ;
#84888=ORIENTED_EDGE ( 'NONE', *, *, #45404, .F. ) ;
#84889=ORIENTED_EDGE ( 'NONE', *, *, #106328, .T. ) ;
#84890=ADVANCED_FACE ( 'NONE', ( #128394 ), #106216, .T. ) ;
#84891=PLANE ( 'NONE',  #83203 ) ;
#84892=DIRECTION ( 'NONE',  ( -0.000000000000000000, 1.000000000000000000, -0.000000000000000000 ) ) ;
#84893=CARTESIAN_POINT ( 'NONE',  ( -3.750000000000025757, 2.500000000000000000, 1.472243186433545459 ) ) ;
#84894=EDGE_CURVE ( 'NONE', #107837, #49056, #35131, .T. ) ;
#84895=ORIENTED_EDGE ( 'NONE', *, *, #74897, .T. ) ;
#84896=ORIENTED_EDGE ( 'NONE', *, *, #37309, .T. ) ;
#84897=EDGE_CURVE ( 'NONE', #78919, #35564, #102011, .T. ) ;
#84898=CARTESIAN_POINT ( 'NONE',  ( -9.350000000000008527, 2.500000000000000000, -6.248780366869521430 ) ) ;
#84899=ADVANCED_FACE ( 'NONE', ( #58993 ), #37362, .T. ) ;
#84900=EDGE_CURVE ( 'NONE', #101832, #9579, #118538, .T. ) ;
#84901=EDGE_LOOP ( 'NONE', ( #40042, #46209, #86502, #5249 ) ) ;
#84902=CARTESIAN_POINT ( 'NONE',  ( -4.150000000000024336, 12.50000000000000000, 1.472243186433545459 ) ) ;
#84903=FACE_OUTER_BOUND ( 'NONE', #102206, .T. ) ;
#84904=VERTEX_POINT ( 'NONE', #8571 ) ;
#84905=DIRECTION ( 'NONE',  ( -0.000000000000000000, -1.000000000000000000, -0.000000000000000000 ) ) ;
#84906=EDGE_CURVE ( 'NONE', #45052, #9793, #49889, .T. ) ;
#84907=LINE ( 'NONE', #113738, #29525 ) ;
#84908=DIRECTION ( 'NONE',  ( 0.000000000000000000, 0.000000000000000000, -1.000000000000000000 ) ) ;
#84909=DIRECTION ( 'NONE',  ( 0.000000000000000000, 0.000000000000000000, 1.000000000000000000 ) ) ;
#84910=ORIENTED_EDGE ( 'NONE', *, *, #33975, .T. ) ;
#84911=ADVANCED_FACE ( 'NONE', ( #106780 ), #64439, .T. ) ;
#84912=DIRECTION ( 'NONE',  ( 0.000000000000000000, -0.000000000000000000, 1.000000000000000000 ) ) ;
#84913=ADVANCED_FACE ( 'NONE', ( #68148 ), #14259, .T. ) ;
#84914=CIRCLE ( 'NONE', #86965, 0.06509327318403745899 ) ;
#84915=AXIS2_PLACEMENT_3D ( 'NONE', #41338, #31499, #42629 ) ;
#84916=CARTESIAN_POINT ( 'NONE',  ( 14.54999999999989591, 2.500000000000000000, 2.165063509461097713 ) ) ;
#84917=EDGE_LOOP ( 'NONE', ( #19809, #44680, #98007, #107709 ) ) ;
#84918=EDGE_LOOP ( 'NONE', ( #46865, #83954 ) ) ;
#84920=DIRECTION ( 'NONE',  ( 0.000000000000000000, -0.9999939076577903929, 0.003490651415223739937 ) ) ;
#84921=DIRECTION ( 'NONE',  ( 0.000000000000000000, 0.000000000000000000, 1.000000000000000000 ) ) ;
#84922=DIRECTION ( 'NONE',  ( 0.000000000000000000, -0.9999939076577903929, 0.003490651415223739937 ) ) ;
#84923=AXIS2_PLACEMENT_3D ( 'NONE', #102350, #79490, #51965 ) ;
#84924=CARTESIAN_POINT ( 'NONE',  ( -0.2000000000000347888, 2.500000000000000000, 0.3464101615137758494 ) ) ;
#84925=CIRCLE ( 'NONE', #74467, 0.09999999999999999167 ) ;
#84926=LINE ( 'NONE', #113757, #126138 ) ;
#84927=DIRECTION ( 'NONE',  ( -0.000000000000000000, -1.000000000000000000, -0.000000000000000000 ) ) ;
#84928=DIRECTION ( 'NONE',  ( -0.000000000000000000, 1.000000000000000000, -0.000000000000000000 ) ) ;
#84929=DIRECTION ( 'NONE',  ( 0.000000000000000000, -0.9999939076577903929, 0.003490651415223739937 ) ) ;
#84930=DIRECTION ( 'NONE',  ( 0.000000000000000000, 0.000000000000000000, 1.000000000000000000 ) ) ;
#84931=AXIS2_PLACEMENT_3D ( 'NONE', #114712, #53872, #74804 ) ;
#84932=CONICAL_SURFACE ( 'NONE', #47384, 0.1000000000000002554, 0.003490658503988666988 ) ;
#84933=VERTEX_POINT ( 'NONE', #87142 ) ;
#84934=VERTEX_POINT ( 'NONE', #7938 ) ;
#84935=ORIENTED_EDGE ( 'NONE', *, *, #56283, .T. ) ;
#84936=ORIENTED_EDGE ( 'NONE', *, *, #91953, .F. ) ;
#84937=FACE_OUTER_BOUND ( 'NONE', #82027, .T. ) ;
#84938=CARTESIAN_POINT ( 'NONE',  ( 9.199999999999915801, 2.500000000000000000, 4.330127018922196314 ) ) ;
#84939=FACE_OUTER_BOUND ( 'NONE', #78154, .T. ) ;
#84940=ORIENTED_EDGE ( 'NONE', *, *, #63545, .T. ) ;
#84941=LINE ( 'NONE', #125507, #107273 ) ;
#84942=DIRECTION ( 'NONE',  ( 0.000000000000000000, 0.000000000000000000, -1.000000000000000000 ) ) ;
#84943=DIRECTION ( 'NONE',  ( 0.000000000000000000, 1.000000000000000000, 0.000000000000000000 ) ) ;
#84944=ORIENTED_EDGE ( 'NONE', *, *, #116754, .T. ) ;
#84945=CARTESIAN_POINT ( 'NONE',  ( 7.099999999999928590, 12.50000000000000000, -5.022947341949754119 ) ) ;
#84946=ORIENTED_EDGE ( 'NONE', *, *, #2702, .T. ) ;
#84947=ADVANCED_FACE ( 'NONE', ( #67487 ), #47890, .T. ) ;
#84948=VECTOR ( 'NONE', #69684, 1000.000000000000000 ) ;
#84949=AXIS2_PLACEMENT_3D ( 'NONE', #106956, #115479, #65749 ) ;
#84950=ORIENTED_EDGE ( 'NONE', *, *, #15380, .T. ) ;
#84951=VERTEX_POINT ( 'NONE', #18413 ) ;
#84952=VERTEX_POINT ( 'NONE', #78645 ) ;
#84953=CARTESIAN_POINT ( 'NONE',  ( 1.249999999999952038, 2.500000000000000000, 5.902370205355745192 ) ) ;
#84954=AXIS2_PLACEMENT_3D ( 'NONE', #16264, #98698, #7749 ) ;
#84955=AXIS2_PLACEMENT_3D ( 'NONE', #63605, #93702, #83870 ) ;
#84956=DIRECTION ( 'NONE',  ( 0.000000000000000000, 0.000000000000000000, 1.000000000000000000 ) ) ;
#84957=FACE_OUTER_BOUND ( 'NONE', #84820, .T. ) ;
#84958=CIRCLE ( 'NONE', #28537, 0.06509327318403745899 ) ;
#84959=CARTESIAN_POINT ( 'NONE',  ( -5.650000000000023448, 2.500000000000000000, -1.818653347947326138 ) ) ;
#84960=ORIENTED_EDGE ( 'NONE', *, *, #73839, .F. ) ;
#84961=VECTOR ( 'NONE', #34641, 1000.000000000000000 ) ;
#84962=DIRECTION ( 'NONE',  ( -0.000000000000000000, -1.000000000000000000, -0.000000000000000000 ) ) ;
#84963=EDGE_LOOP ( 'NONE', ( #13794, #9381 ) ) ;
#84964=CARTESIAN_POINT ( 'NONE',  ( 26.61818291011036308, -2.722754637270933475, -4.358315985290887262 ) ) ;
#84965=CARTESIAN_POINT ( 'NONE',  ( 3.710216157338390275, -1.500000000001404432, -9.999999999999998224 ) ) ;
#84966=PLANE ( 'NONE',  #8781 ) ;
#84967=CARTESIAN_POINT ( 'NONE',  ( -3.150000000000030553, 2.500000000000000000, 6.148780366869520009 ) ) ;
#84968=CIRCLE ( 'NONE', #45274, 0.1000000000000002554 ) ;
#84969=EDGE_LOOP ( 'NONE', ( #121387, #72197, #1506, #29689 ) ) ;
#84970=CIRCLE ( 'NONE', #80793, 0.1000000000000002554 ) ;
#84971=ORIENTED_EDGE ( 'NONE', *, *, #8066, .F. ) ;
#84972=ORIENTED_EDGE ( 'NONE', *, *, #118086, .T. ) ;
#84973=DIRECTION ( 'NONE',  ( -0.000000000000000000, -1.000000000000000000, -0.000000000000000000 ) ) ;
#84974=CARTESIAN_POINT ( 'NONE',  ( -9.600000000000006750, 2.500000000000000000, 0.7928203230275495672 ) ) ;
#84975=DIRECTION ( 'NONE',  ( 0.000000000000000000, 0.000000000000000000, -1.000000000000000000 ) ) ;
#84976=FACE_BOUND ( 'NONE', #82472, .T. ) ;
#84977=LINE ( 'NONE', #16850, #76572 ) ;
#84978=DIRECTION ( 'NONE',  ( 0.000000000000000000, 0.000000000000000000, -1.000000000000000000 ) ) ;
#84979=DIRECTION ( 'NONE',  ( 1.000000000000000000, 0.000000000000000000, 0.000000000000000000 ) ) ;
#84980=CARTESIAN_POINT ( 'NONE',  ( -1.050000000000038680, 12.50000000000000000, 2.576566944158910744 ) ) ;
#84981=CARTESIAN_POINT ( 'NONE',  ( -6.050000000000017586, 2.500000000000000000, 1.818653347947321475 ) ) ;
#84982=FACE_OUTER_BOUND ( 'NONE', #2819, .T. ) ;
#84983=EDGE_LOOP ( 'NONE', ( #59103, #22017 ) ) ;
#84984=EDGE_CURVE ( 'NONE', #94668, #23121, #48523, .T. ) ;
#84985=FACE_OUTER_BOUND ( 'NONE', #74589, .T. ) ;
#84986=ORIENTED_EDGE ( 'NONE', *, *, #19223, .F. ) ;
#84987=ORIENTED_EDGE ( 'NONE', *, *, #103963, .F. ) ;
#84989=ORIENTED_EDGE ( 'NONE', *, *, #42682, .F. ) ;
#84990=EDGE_CURVE ( 'NONE', #6208, #24462, #16386, .T. ) ;
#84991=CARTESIAN_POINT ( 'NONE',  ( -11.24999999999999822, 2.500000000000000000, 5.802370205355744659 ) ) ;
#84992=FACE_BOUND ( 'NONE', #63641, .T. ) ;
#84993=ADVANCED_FACE ( 'NONE', ( #19709 ), #53985, .T. ) ;
#84994=DIRECTION ( 'NONE',  ( 0.000000000000000000, 0.000000000000000000, -1.000000000000000000 ) ) ;
#84995=CIRCLE ( 'NONE', #80810, 0.06509327318403741736 ) ;
#84997=EDGE_CURVE ( 'NONE', #61622, #23744, #43626, .T. ) ;
#84998=ADVANCED_FACE ( 'NONE', ( #116605 ), #26950, .T. ) ;
#84999=EDGE_LOOP ( 'NONE', ( #100111, #86647 ) ) ;
#85000=FACE_OUTER_BOUND ( 'NONE', #106156, .T. ) ;
#85001=EDGE_CURVE ( 'NONE', #115300, #91287, #97888, .T. ) ;
#85002=LINE ( 'NONE', #44442, #41660 ) ;
#85003=ADVANCED_FACE ( 'NONE', ( #111964 ), #110028, .T. ) ;
#85004=VERTEX_POINT ( 'NONE', #32774 ) ;
#85005=CARTESIAN_POINT ( 'NONE',  ( -8.100000000000013856, 12.50000000000000000, -3.983716857408426293 ) ) ;
#85006=CARTESIAN_POINT ( 'NONE',  ( -4.350000000000027178, 12.50000000000000000, -6.906693963081115051 ) ) ;
#85007=VECTOR ( 'NONE', #102195, 1000.000000000000000 ) ;
#85008=ORIENTED_EDGE ( 'NONE', *, *, #95210, .T. ) ;
#85009=CARTESIAN_POINT ( 'NONE',  ( 3.549999999999944755, 2.500000000000000000, -6.841600689897077814 ) ) ;
#85010=DIRECTION ( 'NONE',  ( -0.000000000000000000, -1.000000000000000000, -0.000000000000000000 ) ) ;
#85011=AXIS2_PLACEMENT_3D ( 'NONE', #54438, #66192, #75363 ) ;
#85012=EDGE_CURVE ( 'NONE', #36022, #49975, #40661, .T. ) ;
#85013=CIRCLE ( 'NONE', #116309, 0.06509327318403745899 ) ;
#85014=AXIS2_PLACEMENT_3D ( 'NONE', #75323, #83227, #103508 ) ;
#85015=ORIENTED_EDGE ( 'NONE', *, *, #99401, .T. ) ;
#85016=AXIS2_PLACEMENT_3D ( 'NONE', #25121, #26425, #66963 ) ;
#85017=CARTESIAN_POINT ( 'NONE',  ( -13.14999999999999147, 2.500000000000000000, -2.411473670974875638 ) ) ;
#85018=DIRECTION ( 'NONE',  ( -0.000000000000000000, 1.000000000000000000, -0.000000000000000000 ) ) ;
#85019=DIRECTION ( 'NONE',  ( 0.000000000000000000, 0.000000000000000000, 1.000000000000000000 ) ) ;
#85020=ORIENTED_EDGE ( 'NONE', *, *, #61233, .T. ) ;
#85021=VERTEX_POINT ( 'NONE', #101495 ) ;
#85022=DIRECTION ( 'NONE',  ( 0.000000000000000000, 0.000000000000000000, 1.000000000000000000 ) ) ;
#85023=VERTEX_POINT ( 'NONE', #62851 ) ;
#85024=DIRECTION ( 'NONE',  ( 0.000000000000000000, 0.000000000000000000, 1.000000000000000000 ) ) ;
#85025=DIRECTION ( 'NONE',  ( 0.000000000000000000, 0.000000000000000000, 1.000000000000000000 ) ) ;
#85026=VERTEX_POINT ( 'NONE', #102761 ) ;
#85027=FACE_OUTER_BOUND ( 'NONE', #34096, .T. ) ;
#85028=DIRECTION ( 'NONE',  ( 0.000000000000000000, 0.000000000000000000, 1.000000000000000000 ) ) ;
#85029=DIRECTION ( 'NONE',  ( -0.000000000000000000, 1.000000000000000000, -0.000000000000000000 ) ) ;
#85030=DIRECTION ( 'NONE',  ( 0.000000000000000000, 1.000000000000000000, 0.000000000000000000 ) ) ;
#85031=EDGE_CURVE ( 'NONE', #107528, #34472, #72861, .T. ) ;
#85032=CIRCLE ( 'NONE', #83007, 0.06509327318403745899 ) ;
#85033=DIRECTION ( 'NONE',  ( 0.000000000000000000, 0.000000000000000000, 1.000000000000000000 ) ) ;
#85034=VECTOR ( 'NONE', #67458, 1000.000000000000000 ) ;
#85035=CONICAL_SURFACE ( 'NONE', #20212, 0.1000000000000002554, 0.003490658503988666988 ) ;
#85037=VERTEX_POINT ( 'NONE', #2622 ) ;
#85038=DIRECTION ( 'NONE',  ( -0.000000000000000000, 1.000000000000000000, -0.000000000000000000 ) ) ;
#85039=AXIS2_PLACEMENT_3D ( 'NONE', #78728, #108794, #38140 ) ;
#85040=CARTESIAN_POINT ( 'NONE',  ( 17.19804440726969474, -0.4677972980984264617, 5.492654682185391657 ) ) ;
#85041=CARTESIAN_POINT ( 'NONE',  ( -7.300000000000018474, 12.50000000000000000, -3.983716857408426293 ) ) ;
#85042=ORIENTED_EDGE ( 'NONE', *, *, #2682, .F. ) ;
#85043=ORIENTED_EDGE ( 'NONE', *, *, #113728, .F. ) ;
#85044=EDGE_LOOP ( 'NONE', ( #7726, #6377 ) ) ;
#85045=ADVANCED_FACE ( 'NONE', ( #11809 ), #5927, .T. ) ;
#85046=CARTESIAN_POINT ( 'NONE',  ( 1.899999999999949507, 12.50000000000000000, 3.983716857408420964 ) ) ;
#85047=AXIS2_PLACEMENT_3D ( 'NONE', #14790, #63282, #94669 ) ;
#85048=ADVANCED_FACE ( 'NONE', ( #54 ), #89583, .T. ) ;
#85049=CONICAL_SURFACE ( 'NONE', #18146, 0.09999999999999999167, 0.003490658503988666988 ) ;
#85050=DIRECTION ( 'NONE',  ( -0.6795087154616696878, -6.363550617825450602E-16, 0.7336674352945151689 ) ) ;
#85051=DIRECTION ( 'NONE',  ( -0.000000000000000000, 1.000000000000000000, -0.000000000000000000 ) ) ;
#85052=VECTOR ( 'NONE', #122481, 1000.000000000000000 ) ;
#85053=EDGE_CURVE ( 'NONE', #122997, #51911, #70100, .T. ) ;
#85055=DIRECTION ( 'NONE',  ( 0.000000000000000000, 0.000000000000000000, -1.000000000000000000 ) ) ;
#85056=CARTESIAN_POINT ( 'NONE',  ( -4.800000000000022915, 12.50000000000000000, -0.4115034346978157509 ) ) ;
#85057=CARTESIAN_POINT ( 'NONE',  ( -3.350000000000028511, 2.500000000000000000, -1.572243186433550211 ) ) ;
#85058=DIRECTION ( 'NONE',  ( 0.000000000000000000, 0.000000000000000000, -1.000000000000000000 ) ) ;
#85059=DIRECTION ( 'NONE',  ( 0.000000000000000000, 0.000000000000000000, 1.000000000000000000 ) ) ;
#85060=AXIS2_PLACEMENT_3D ( 'NONE', #63480, #92948, #103406 ) ;
#85061=EDGE_CURVE ( 'NONE', #16079, #48393, #112605, .T. ) ;
#85062=DIRECTION ( 'NONE',  ( 0.000000000000000000, 1.000000000000000000, 0.000000000000000000 ) ) ;
#85063=AXIS2_PLACEMENT_3D ( 'NONE', #13171, #62936, #3372 ) ;
#85064=EDGE_CURVE ( 'NONE', #108831, #8397, #22937, .T. ) ;
#85066=ORIENTED_EDGE ( 'NONE', *, *, #41477, .T. ) ;
#85067=AXIS2_PLACEMENT_3D ( 'NONE', #22624, #63164, #112283 ) ;
#85068=CIRCLE ( 'NONE', #26499, 0.06509327318403745899 ) ;
#85069=ADVANCED_FACE ( 'NONE', ( #121125 ), #41494, .T. ) ;
#85070=CARTESIAN_POINT ( 'NONE',  ( 12.69999999999989804, 2.500000000000000000, 0.4464101615137735513 ) ) ;
#85071=ORIENTED_EDGE ( 'NONE', *, *, #30060, .F. ) ;
#85072=ORIENTED_EDGE ( 'NONE', *, *, #98026, .T. ) ;
#85073=DIRECTION ( 'NONE',  ( -0.000000000000000000, 1.000000000000000000, -0.000000000000000000 ) ) ;
#85074=DIRECTION ( 'NONE',  ( 0.000000000000000000, 0.000000000000000000, 1.000000000000000000 ) ) ;
#85075=DIRECTION ( 'NONE',  ( 0.000000000000000000, 0.000000000000000000, -1.000000000000000000 ) ) ;
#85076=ADVANCED_FACE ( 'NONE', ( #72038 ), #102137, .T. ) ;
#85077=CARTESIAN_POINT ( 'NONE',  ( -0.2000000000000412836, 2.500000000000000000, 4.776537180435972196 ) ) ;
#85078=CARTESIAN_POINT ( 'NONE',  ( -1.850000000000033840, 2.500000000000000000, 6.841600689897072485 ) ) ;
#85079=CARTESIAN_POINT ( 'NONE',  ( 2.049999999999948308, 12.50000000000000000, 6.495190528383297135 ) ) ;
#85080=DIRECTION ( 'NONE',  ( -0.000000000000000000, -1.000000000000000000, -0.000000000000000000 ) ) ;
#85081=ORIENTED_EDGE ( 'NONE', *, *, #38638, .F. ) ;
#85082=DIRECTION ( 'NONE',  ( 0.000000000000000000, 0.000000000000000000, -1.000000000000000000 ) ) ;
#85083=AXIS2_PLACEMENT_3D ( 'NONE', #78302, #28545, #36448 ) ;
#85084=CARTESIAN_POINT ( 'NONE',  ( 1.849999999999949019, 2.500000000000000000, 6.741600689897071952 ) ) ;
#85085=ORIENTED_EDGE ( 'NONE', *, *, #93874, .F. ) ;
#85086=ORIENTED_EDGE ( 'NONE', *, *, #64650, .T. ) ;
#85087=ORIENTED_EDGE ( 'NONE', *, *, #54244, .T. ) ;
#85088=ORIENTED_EDGE ( 'NONE', *, *, #23768, .T. ) ;
#85089=DIRECTION ( 'NONE',  ( 0.000000000000000000, -0.000000000000000000, 1.000000000000000000 ) ) ;
#85090=DIRECTION ( 'NONE',  ( -0.000000000000000000, 1.000000000000000000, -0.000000000000000000 ) ) ;
#85091=CONICAL_SURFACE ( 'NONE', #116478, 0.1000000000000002554, 0.003490658503988666988 ) ;
#85092=DIRECTION ( 'NONE',  ( -0.000000000000000000, 1.000000000000000000, -0.000000000000000000 ) ) ;
#85093=CONICAL_SURFACE ( 'NONE', #87149, 0.09999999999999982514, 0.003490658503988666988 ) ;
#85094=CARTESIAN_POINT ( 'NONE',  ( -5.850000000000018296, 2.500000000000000000, 2.957883832488649389 ) ) ;
#85095=LINE ( 'NONE', #15037, #11593 ) ;
#85096=EDGE_LOOP ( 'NONE', ( #115202, #63136 ) ) ;
#85097=CARTESIAN_POINT ( 'NONE',  ( -12.04999999999999538, 2.500000000000000000, 6.495190528383297135 ) ) ;
#85098=CARTESIAN_POINT ( 'NONE',  ( 6.649999999999927525, 2.500000000000000000, 2.165063509461097713 ) ) ;
#85099=CIRCLE ( 'NONE', #9801, 0.06509327318403745899 ) ;
#85100=CIRCLE ( 'NONE', #1475, 0.06509327318403745899 ) ;
#85101=DIRECTION ( 'NONE',  ( 0.000000000000000000, 0.000000000000000000, 1.000000000000000000 ) ) ;
#85102=EDGE_LOOP ( 'NONE', ( #100052, #103301, #2705, #105003 ) ) ;
#85103=ADVANCED_FACE ( 'NONE', ( #20989 ), #700, .T. ) ;
#85104=EDGE_LOOP ( 'NONE', ( #31707, #63367 ) ) ;
#85105=ORIENTED_EDGE ( 'NONE', *, *, #9898, .T. ) ;
#85106=DIRECTION ( 'NONE',  ( 0.000000000000000000, 0.000000000000000000, 1.000000000000000000 ) ) ;
#85107=CONICAL_SURFACE ( 'NONE', #45417, 0.1000000000000000056, 0.003490658503988666988 ) ;
#85108=DIRECTION ( 'NONE',  ( 0.000000000000000000, 1.000000000000000000, 0.000000000000000000 ) ) ;
#85109=DIRECTION ( 'NONE',  ( -0.000000000000000000, -1.000000000000000000, -0.000000000000000000 ) ) ;
#85110=CONICAL_SURFACE ( 'NONE', #68481, 0.1000000000000002554, 0.003490658503988666988 ) ;
#85111=ORIENTED_EDGE ( 'NONE', *, *, #79504, .T. ) ;
#85112=FACE_OUTER_BOUND ( 'NONE', #78044, .T. ) ;
#85113=DIRECTION ( 'NONE',  ( -4.274815082592931898E-19, -0.9999939076577903929, -0.003490651415223739937 ) ) ;
#85114=ADVANCED_FACE ( 'NONE', ( #50448 ), #120483, .T. ) ;
#85115=DIRECTION ( 'NONE',  ( -0.000000000000000000, -1.000000000000000000, -0.000000000000000000 ) ) ;
#85116=CARTESIAN_POINT ( 'NONE',  ( -6.249999999999984901, 12.50000000000000000, -6.495190528383302464 ) ) ;
#85117=DIRECTION ( 'NONE',  ( 0.000000000000000000, 0.000000000000000000, -1.000000000000000000 ) ) ;
#85118=ORIENTED_EDGE ( 'NONE', *, *, #19014, .F. ) ;
#85120=ORIENTED_EDGE ( 'NONE', *, *, #71655, .F. ) ;
#85121=ORIENTED_EDGE ( 'NONE', *, *, #73497, .F. ) ;
#85122=VERTEX_POINT ( 'NONE', #60914 ) ;
#85123=CARTESIAN_POINT ( 'NONE',  ( 8.749999999999921840, 2.500000000000000000, 2.857883832488649301 ) ) ;
#85124=FACE_BOUND ( 'NONE', #41914, .T. ) ;
#85125=AXIS2_PLACEMENT_3D ( 'NONE', #30806, #38703, #109341 ) ;
#85126=CARTESIAN_POINT ( 'NONE',  ( 10.64999999999991331, 12.50000000000000000, -1.753560074763288457 ) ) ;
#85127=CARTESIAN_POINT ( 'NONE',  ( 11.24999999999990763, 12.50000000000000000, 1.537336459617582918 ) ) ;
#85128=CONICAL_SURFACE ( 'NONE', #37028, 0.09999999999999982514, 0.003490658503988666988 ) ;
#85129=DIRECTION ( 'NONE',  ( 0.000000000000000000, 0.000000000000000000, -1.000000000000000000 ) ) ;
#85130=VECTOR ( 'NONE', #112176, 1000.000000000000000 ) ;
#85131=VERTEX_POINT ( 'NONE', #11161 ) ;
#85132=CARTESIAN_POINT ( 'NONE',  ( 6.899999999999926636, 12.50000000000000000, -0.3464101615137782364 ) ) ;
#85133=DIRECTION ( 'NONE',  ( -0.000000000000000000, 1.000000000000000000, -0.000000000000000000 ) ) ;
#85134=CIRCLE ( 'NONE', #114382, 0.06509327318403745899 ) ;
#85135=FACE_OUTER_BOUND ( 'NONE', #5869, .T. ) ;
#85136=VECTOR ( 'NONE', #107060, 1000.000000000000000 ) ;
#85137=DIRECTION ( 'NONE',  ( -4.274815082592931898E-19, -0.9999939076577903929, -0.003490651415223739937 ) ) ;
#85138=EDGE_LOOP ( 'NONE', ( #121054, #90168 ) ) ;
#85139=LINE ( 'NONE', #14453, #19691 ) ;
#85140=CONICAL_SURFACE ( 'NONE', #62180, 0.1000000000000002554, 0.003490658503988666988 ) ;
#85142=EDGE_CURVE ( 'NONE', #104830, #31947, #91632, .T. ) ;
#85143=FACE_OUTER_BOUND ( 'NONE', #60633, .T. ) ;
#85144=ORIENTED_EDGE ( 'NONE', *, *, #47825, .F. ) ;
#85145=CARTESIAN_POINT ( 'NONE',  ( 3.299999999999944755, 2.500000000000000000, -4.430127018922202176 ) ) ;
#85146=AXIS2_PLACEMENT_3D ( 'NONE', #33241, #102591, #50938 ) ;
#85147=VERTEX_POINT ( 'NONE', #41936 ) ;
#85148=FACE_BOUND ( 'NONE', #22183, .T. ) ;
#85149=ADVANCED_FACE ( 'NONE', ( #95540 ), #85703, .T. ) ;
#85150=FACE_OUTER_BOUND ( 'NONE', #125112, .T. ) ;
#85151=CONICAL_SURFACE ( 'NONE', #87204, 0.1000000000000000472, 0.003490658503988666988 ) ;
#85152=CONICAL_SURFACE ( 'NONE', #89374, 0.09999999999999982514, 0.003490658503988666988 ) ;
#85153=ORIENTED_EDGE ( 'NONE', *, *, #49751, .T. ) ;
#85154=DIRECTION ( 'NONE',  ( -4.274815082592931898E-19, -0.9999939076577903929, -0.003490651415223739937 ) ) ;
#85155=DIRECTION ( 'NONE',  ( 0.000000000000000000, 1.000000000000000000, 0.000000000000000000 ) ) ;
#85156=ADVANCED_FACE ( 'NONE', ( #73961 ), #1734, .T. ) ;
#85157=VERTEX_POINT ( 'NONE', #93598 ) ;
#85158=ADVANCED_FACE ( 'NONE', ( #105999 ), #33411, .T. ) ;
#85159=EDGE_LOOP ( 'NONE', ( #57117, #16910 ) ) ;
#85160=EDGE_CURVE ( 'NONE', #33313, #112742, #54321, .T. ) ;
#85163=ORIENTED_EDGE ( 'NONE', *, *, #19555, .F. ) ;
#85165=DIRECTION ( 'NONE',  ( -0.000000000000000000, -1.000000000000000000, -0.000000000000000000 ) ) ;
#85166=CARTESIAN_POINT ( 'NONE',  ( -0.8500000000000386136, 2.500000000000000000, 2.857883832488649301 ) ) ;
#85167=CARTESIAN_POINT ( 'NONE',  ( 1.899999999999949507, 2.500000000000000000, 3.983716857408420964 ) ) ;
#85168=FACE_OUTER_BOUND ( 'NONE', #12183, .T. ) ;
#85169=CARTESIAN_POINT ( 'NONE',  ( 11.24999999999990763, 2.500000000000000000, 1.572243186433545548 ) ) ;
#85170=CIRCLE ( 'NONE', #122832, 0.1000000000000000472 ) ;
#85171=EDGE_CURVE ( 'NONE', #74962, #85395, #83336, .T. ) ;
#85172=EDGE_CURVE ( 'NONE', #110704, #46732, #85372, .T. ) ;
#85173=ADVANCED_FACE ( 'NONE', ( #105355 ), #125082, .T. ) ;
#85175=ORIENTED_EDGE ( 'NONE', *, *, #84847, .T. ) ;
#85176=CARTESIAN_POINT ( 'NONE',  ( 9.149999999999920419, 2.500000000000000000, -5.802370205355749988 ) ) ;
#85177=DIRECTION ( 'NONE',  ( -4.274815082592931898E-19, -0.9999939076577903929, -0.003490651415223739937 ) ) ;
#85178=DIRECTION ( 'NONE',  ( 0.000000000000000000, 1.000000000000000000, 0.000000000000000000 ) ) ;
#85179=CARTESIAN_POINT ( 'NONE',  ( -2.300000000000033129, 12.50000000000000000, 3.983716857408420076 ) ) ;
#85180=ORIENTED_EDGE ( 'NONE', *, *, #79725, .F. ) ;
#85181=EDGE_LOOP ( 'NONE', ( #87088, #9532 ) ) ;
#85182=FACE_BOUND ( 'NONE', #80004, .T. ) ;
#85183=EDGE_LOOP ( 'NONE', ( #48306, #61862, #124225, #111979 ) ) ;
#85184=DIRECTION ( 'NONE',  ( -0.000000000000000000, -1.000000000000000000, -0.000000000000000000 ) ) ;
#85185=FACE_OUTER_BOUND ( 'NONE', #111314, .T. ) ;
#85186=EDGE_LOOP ( 'NONE', ( #99572, #14184, #50876, #12514 ) ) ;
#85187=DIRECTION ( 'NONE',  ( -0.000000000000000000, 1.000000000000000000, -0.000000000000000000 ) ) ;
#85188=CARTESIAN_POINT ( 'NONE',  ( -2.700000000000030820, 2.500000000000000000, -3.983716857408426293 ) ) ;
#85189=CIRCLE ( 'NONE', #66403, 0.1000000000000002554 ) ;
#85190=CARTESIAN_POINT ( 'NONE',  ( 11.64999999999990266, 12.50000000000000000, -6.495190528383302464 ) ) ;
#85191=CONICAL_SURFACE ( 'NONE', #51753, 0.1000000000000002554, 0.003490658503988666988 ) ;
#85192=PLANE ( 'NONE',  #602 ) ;
#85193=CARTESIAN_POINT ( 'NONE',  ( -14.19999999999998685, 2.500000000000000000, 0.09999999999999989453 ) ) ;
#85194=CARTESIAN_POINT ( 'NONE',  ( 13.94999999999989448, 2.500000000000000000, -2.611473670974877592 ) ) ;
#85195=DIRECTION ( 'NONE',  ( 0.000000000000000000, 0.000000000000000000, 1.000000000000000000 ) ) ;
#85196=DIRECTION ( 'NONE',  ( 0.000000000000000000, 1.000000000000000000, 0.000000000000000000 ) ) ;
#85197=VECTOR ( 'NONE', #112507, 1000.000000000000000 ) ;
#85198=ORIENTED_EDGE ( 'NONE', *, *, #45661, .F. ) ;
#85199=CIRCLE ( 'NONE', #28782, 0.06509327318403741736 ) ;
#85200=EDGE_LOOP ( 'NONE', ( #45091, #51415, #91617, #114160 ) ) ;
#85201=DIRECTION ( 'NONE',  ( -4.274815082592931898E-19, -0.9999939076577903929, -0.003490651415223739937 ) ) ;
#85202=ORIENTED_EDGE ( 'NONE', *, *, #64235, .T. ) ;
#85203=DIRECTION ( 'NONE',  ( -0.000000000000000000, 1.000000000000000000, -0.000000000000000000 ) ) ;
#85204=VERTEX_POINT ( 'NONE', #124992 ) ;
#85205=ORIENTED_EDGE ( 'NONE', *, *, #65212, .T. ) ;
#85206=ORIENTED_EDGE ( 'NONE', *, *, #103206, .F. ) ;
#85207=CARTESIAN_POINT ( 'NONE',  ( -3.550000000000027356, 12.50000000000000000, -2.446380397790840266 ) ) ;
#85208=AXIS2_PLACEMENT_3D ( 'NONE', #61693, #10613, #101611 ) ;
#85209=DIRECTION ( 'NONE',  ( 0.000000000000000000, 0.000000000000000000, -1.000000000000000000 ) ) ;
#85211=DIRECTION ( 'NONE',  ( 0.000000000000000000, -0.000000000000000000, 1.000000000000000000 ) ) ;
#85212=DIRECTION ( 'NONE',  ( 0.000000000000000000, -0.9999939076577903929, 0.003490651415223739937 ) ) ;
#85213=DIRECTION ( 'NONE',  ( 0.000000000000000000, 0.000000000000000000, 1.000000000000000000 ) ) ;
#85214=VECTOR ( 'NONE', #78986, 1000.000000000000000 ) ;
#85215=EDGE_LOOP ( 'NONE', ( #86022, #128826 ) ) ;
#85216=ADVANCED_FACE ( 'NONE', ( #103424 ), #13734, .T. ) ;
#85217=DIRECTION ( 'NONE',  ( 0.000000000000000000, 0.000000000000000000, 1.000000000000000000 ) ) ;
#85218=VERTEX_POINT ( 'NONE', #114514 ) ;
#85219=ADVANCED_FACE ( 'NONE', ( #24861 ), #64133, .T. ) ;
#85220=CIRCLE ( 'NONE', #51778, 0.1000000000000000472 ) ;
#85221=ORIENTED_EDGE ( 'NONE', *, *, #110569, .F. ) ;
#85222=ORIENTED_EDGE ( 'NONE', *, *, #29533, .F. ) ;
#85223=EDGE_CURVE ( 'NONE', #27204, #37524, #79132, .T. ) ;
#85224=CIRCLE ( 'NONE', #45527, 0.09999999999999982514 ) ;
#85225=PLANE ( 'NONE',  #107034 ) ;
#85226=EDGE_LOOP ( 'NONE', ( #35788, #25545 ) ) ;
#85227=ORIENTED_EDGE ( 'NONE', *, *, #5232, .T. ) ;
#85228=ORIENTED_EDGE ( 'NONE', *, *, #72619, .T. ) ;
#85229=CIRCLE ( 'NONE', #60120, 0.1000000000000000472 ) ;
#85230=AXIS2_PLACEMENT_3D ( 'NONE', #12423, #52358, #92271 ) ;
#85231=DIRECTION ( 'NONE',  ( 0.000000000000000000, 0.000000000000000000, -1.000000000000000000 ) ) ;
#85232=EDGE_CURVE ( 'NONE', #106006, #73789, #34038, .T. ) ;
#85233=CARTESIAN_POINT ( 'NONE',  ( 1.249999999999953815, 12.50000000000000000, 1.472243186433545459 ) ) ;
#85234=DIRECTION ( 'NONE',  ( 0.000000000000000000, 0.000000000000000000, 1.000000000000000000 ) ) ;
#85235=CIRCLE ( 'NONE', #24694, 0.06509327318403745899 ) ;
#85236=CARTESIAN_POINT ( 'NONE',  ( -9.800000000000007816, 12.50000000000000000, -3.983716857408421852 ) ) ;
#85237=CARTESIAN_POINT ( 'NONE',  ( -5.850000000000019185, 2.500000000000000000, 6.395190528383296602 ) ) ;
#85238=DIRECTION ( 'NONE',  ( 0.000000000000000000, -0.000000000000000000, 1.000000000000000000 ) ) ;
#85239=EDGE_LOOP ( 'NONE', ( #111768, #8681, #30313, #11540 ) ) ;
#85240=AXIS2_PLACEMENT_3D ( 'NONE', #99038, #21113, #110780 ) ;
#85241=CARTESIAN_POINT ( 'NONE',  ( 11.44999999999991047, 12.50000000000000000, -2.511473670974877948 ) ) ;
#85242=AXIS2_PLACEMENT_3D ( 'NONE', #121405, #101777, #52038 ) ;
#85243=ORIENTED_EDGE ( 'NONE', *, *, #48750, .T. ) ;
#85244=AXIS2_PLACEMENT_3D ( 'NONE', #70967, #22536, #110878 ) ;
#85245=DIRECTION ( 'NONE',  ( 0.000000000000000000, -0.000000000000000000, 1.000000000000000000 ) ) ;
#85246=ORIENTED_EDGE ( 'NONE', *, *, #64738, .F. ) ;
#85247=CARTESIAN_POINT ( 'NONE',  ( 7.099999999999928590, 2.500000000000000000, -5.122947341949753763 ) ) ;
#85248=ORIENTED_EDGE ( 'NONE', *, *, #61075, .F. ) ;
#85249=AXIS2_PLACEMENT_3D ( 'NONE', #36461, #76373, #94073 ) ;
#85250=EDGE_CURVE ( 'NONE', #101710, #63288, #85458, .T. ) ;
#85251=ORIENTED_EDGE ( 'NONE', *, *, #20288, .F. ) ;
#85252=PLANE ( 'NONE',  #9376 ) ;
#85253=CARTESIAN_POINT ( 'NONE',  ( 14.59999999999989484, 2.500000000000000000, -0.5928203230275541635 ) ) ;
#85254=AXIS2_PLACEMENT_3D ( 'NONE', #4087, #45968, #45325 ) ;
#85255=VECTOR ( 'NONE', #47306, 1000.000000000000000 ) ;
#85256=CARTESIAN_POINT ( 'NONE',  ( -6.050000000000020250, 2.500000000000000000, -2.511473670974877948 ) ) ;
#85257=LINE ( 'NONE', #36169, #26179 ) ;
#85258=ORIENTED_EDGE ( 'NONE', *, *, #66760, .F. ) ;
#85259=DIRECTION ( 'NONE',  ( 0.000000000000000000, 1.000000000000000000, 0.000000000000000000 ) ) ;
#85260=DIRECTION ( 'NONE',  ( -0.000000000000000000, -1.000000000000000000, -0.000000000000000000 ) ) ;
#85261=PLANE ( 'NONE',  #106638 ) ;
#85262=DIRECTION ( 'NONE',  ( 0.000000000000000000, 0.000000000000000000, -1.000000000000000000 ) ) ;
#85263=DIRECTION ( 'NONE',  ( 0.000000000000000000, 0.000000000000000000, -1.000000000000000000 ) ) ;
#85264=EDGE_LOOP ( 'NONE', ( #2802, #98190, #48148, #42304 ) ) ;
#85265=EDGE_CURVE ( 'NONE', #71725, #126533, #35970, .T. ) ;
#85266=ORIENTED_EDGE ( 'NONE', *, *, #47238, .T. ) ;
#85267=ORIENTED_EDGE ( 'NONE', *, *, #29345, .T. ) ;
#85268=DIRECTION ( 'NONE',  ( 0.000000000000000000, 0.000000000000000000, 1.000000000000000000 ) ) ;
#85269=DIRECTION ( 'NONE',  ( 0.000000000000000000, 0.000000000000000000, 1.000000000000000000 ) ) ;
#85270=CIRCLE ( 'NONE', #35125, 0.1000000000000002554 ) ;
#85272=FACE_OUTER_BOUND ( 'NONE', #126962, .T. ) ;
#85273=DIRECTION ( 'NONE',  ( -0.000000000000000000, -1.000000000000000000, -0.000000000000000000 ) ) ;
#85274=EDGE_CURVE ( 'NONE', #112496, #26891, #70795, .T. ) ;
#85275=CARTESIAN_POINT ( 'NONE',  ( -4.250072516143177381E-14, 2.500000000000000000, -3.637306695894650055 ) ) ;
#85276=CARTESIAN_POINT ( 'NONE',  ( 11.84999999999990372, 2.500000000000000000, -6.741600689897078169 ) ) ;
#85277=ORIENTED_EDGE ( 'NONE', *, *, #75378, .T. ) ;
#85278=AXIS2_PLACEMENT_3D ( 'NONE', #55121, #53827, #93757 ) ;
#85279=AXIS2_PLACEMENT_3D ( 'NONE', #26372, #116667, #115355 ) ;
#85280=CARTESIAN_POINT ( 'NONE',  ( 0.8499999999999545697, 2.500000000000000000, -1.472243186433550122 ) ) ;
#85281=CARTESIAN_POINT ( 'NONE',  ( -12.04999999999999538, 12.50000000000000000, 6.560283801567334372 ) ) ;
#85282=ORIENTED_EDGE ( 'NONE', *, *, #6961, .F. ) ;
#85283=EDGE_CURVE ( 'NONE', #62002, #95428, #70897, .T. ) ;
#85284=DIRECTION ( 'NONE',  ( 0.000000000000000000, 1.000000000000000000, 0.000000000000000000 ) ) ;
#85285=CARTESIAN_POINT ( 'NONE',  ( 10.44999999999991047, 12.50000000000000000, 2.165063509461097713 ) ) ;
#85286=CONICAL_SURFACE ( 'NONE', #49716, 0.1000000000000002554, 0.003490658503988666988 ) ;
#85287=DIRECTION ( 'NONE',  ( 0.000000000000000000, 0.000000000000000000, -1.000000000000000000 ) ) ;
#85288=CONICAL_SURFACE ( 'NONE', #116678, 0.1000000000000000472, 0.003490658503988666988 ) ;
#85289=ORIENTED_EDGE ( 'NONE', *, *, #45463, .F. ) ;
#85290=DIRECTION ( 'NONE',  ( 0.000000000000000000, -0.9999939076577903929, 0.003490651415223739937 ) ) ;
#85291=ORIENTED_EDGE ( 'NONE', *, *, #125096, .T. ) ;
#85292=FACE_OUTER_BOUND ( 'NONE', #44323, .T. ) ;
#85293=FACE_OUTER_BOUND ( 'NONE', #47229, .T. ) ;
#85294=ORIENTED_EDGE ( 'NONE', *, *, #107796, .F. ) ;
#85295=DIRECTION ( 'NONE',  ( 0.000000000000000000, 1.000000000000000000, 0.000000000000000000 ) ) ;
#85296=ADVANCED_FACE ( 'NONE', ( #115811 ), #87505, .T. ) ;
#85297=CARTESIAN_POINT ( 'NONE',  ( -1.900000000000034106, 2.500000000000000000, 0.3464101615137735735 ) ) ;
#85298=AXIS2_PLACEMENT_3D ( 'NONE', #36967, #38260, #19231 ) ;
#85299=ORIENTED_EDGE ( 'NONE', *, *, #66115, .F. ) ;
#85300=DIRECTION ( 'NONE',  ( 0.000000000000000000, 0.000000000000000000, -1.000000000000000000 ) ) ;
#85301=EDGE_CURVE ( 'NONE', #87786, #94540, #117085, .T. ) ;
#85302=AXIS2_PLACEMENT_3D ( 'NONE', #62298, #121196, #79360 ) ;
#85303=ORIENTED_EDGE ( 'NONE', *, *, #10020, .T. ) ;
#85304=VERTEX_POINT ( 'NONE', #58833 ) ;
#85305=AXIS2_PLACEMENT_3D ( 'NONE', #19181, #62370, #100986 ) ;
#85306=PLANE ( 'NONE',  #27517 ) ;
#85307=CARTESIAN_POINT ( 'NONE',  ( -1.250000000000036193, 12.50000000000000000, 5.802370205355744659 ) ) ;
#85308=EDGE_CURVE ( 'NONE', #117873, #89637, #14433, .T. ) ;
#85309=EDGE_CURVE ( 'NONE', #124116, #47422, #58290, .T. ) ;
#85310=ORIENTED_EDGE ( 'NONE', *, *, #985, .T. ) ;
#85311=EDGE_CURVE ( 'NONE', #24620, #124866, #100145, .T. ) ;
#85312=AXIS2_PLACEMENT_3D ( 'NONE', #72193, #72827, #4070 ) ;
#85313=EDGE_CURVE ( 'NONE', #29034, #126026, #9081, .T. ) ;
#85314=CARTESIAN_POINT ( 'NONE',  ( -15.39999999999997904, 12.50000000000000000, -0.6928203230275519209 ) ) ;
#85315=DIRECTION ( 'NONE',  ( -0.000000000000000000, 1.000000000000000000, -0.000000000000000000 ) ) ;
#85316=AXIS2_PLACEMENT_3D ( 'NONE', #102754, #72671, #43223 ) ;
#85317=EDGE_LOOP ( 'NONE', ( #19077, #81602, #127193, #72661 ) ) ;
#85318=CARTESIAN_POINT ( 'NONE',  ( -12.89999999999999147, 12.50000000000000000, -0.6928203230275500335 ) ) ;
#85319=DIRECTION ( 'NONE',  ( -0.000000000000000000, -1.000000000000000000, -0.000000000000000000 ) ) ;
#85320=EDGE_CURVE ( 'NONE', #45027, #6696, #16303, .T. ) ;
#85321=DIRECTION ( 'NONE',  ( -0.000000000000000000, -1.000000000000000000, -0.000000000000000000 ) ) ;
#85322=DIRECTION ( 'NONE',  ( 0.000000000000000000, 0.000000000000000000, -1.000000000000000000 ) ) ;
#85323=EDGE_CURVE ( 'NONE', #66996, #1899, #114704, .T. ) ;
#85324=DIRECTION ( 'NONE',  ( 0.000000000000000000, 1.000000000000000000, 0.000000000000000000 ) ) ;
#85325=CONICAL_SURFACE ( 'NONE', #1411, 0.09999999999999982514, 0.003490658503988666988 ) ;
#85326=DIRECTION ( 'NONE',  ( 0.000000000000000000, -0.9999939076577903929, 0.003490651415223739937 ) ) ;
#85327=EDGE_CURVE ( 'NONE', #25449, #95824, #60455, .T. ) ;
#85329=EDGE_CURVE ( 'NONE', #78151, #16115, #128889, .T. ) ;
#85330=EDGE_LOOP ( 'NONE', ( #110083, #101526, #1497, #94453 ) ) ;
#85331=VERTEX_POINT ( 'NONE', #16929 ) ;
#85332=VERTEX_POINT ( 'NONE', #47092 ) ;
#85333=ORIENTED_EDGE ( 'NONE', *, *, #102502, .T. ) ;
#85334=DIRECTION ( 'NONE',  ( 0.000000000000000000, 1.000000000000000000, 0.000000000000000000 ) ) ;
#85336=CARTESIAN_POINT ( 'NONE',  ( -6.650000000000018119, 2.500000000000000000, -6.595190528383302109 ) ) ;
#85337=VECTOR ( 'NONE', #51212, 1000.000000000000000 ) ;
#85338=VERTEX_POINT ( 'NONE', #106636 ) ;
#85339=FACE_BOUND ( 'NONE', #59619, .T. ) ;
#85340=ADVANCED_FACE ( 'NONE', ( #79129 ), #1835, .T. ) ;
#85341=DIRECTION ( 'NONE',  ( 0.000000000000000000, 0.000000000000000000, 1.000000000000000000 ) ) ;
#85342=DIRECTION ( 'NONE',  ( 0.000000000000000000, -0.9999939076577903929, 0.003490651415223739937 ) ) ;
#85343=DIRECTION ( 'NONE',  ( 0.000000000000000000, 0.000000000000000000, -1.000000000000000000 ) ) ;
#85344=CONICAL_SURFACE ( 'NONE', #110380, 0.1000000000000002554, 0.003490658503988666988 ) ;
#85345=AXIS2_PLACEMENT_3D ( 'NONE', #24282, #2049, #21711 ) ;
#85346=DIRECTION ( 'NONE',  ( 0.000000000000000000, 0.000000000000000000, 1.000000000000000000 ) ) ;
#85347=DIRECTION ( 'NONE',  ( -0.000000000000000000, 1.000000000000000000, -0.000000000000000000 ) ) ;
#85348=LINE ( 'NONE', #104965, #1602 ) ;
#85349=LINE ( 'NONE', #15943, #55877 ) ;
#85350=DIRECTION ( 'NONE',  ( -0.000000000000000000, -1.000000000000000000, -0.000000000000000000 ) ) ;
#85351=DIRECTION ( 'NONE',  ( 0.000000000000000000, 0.000000000000000000, -1.000000000000000000 ) ) ;
#85352=CARTESIAN_POINT ( 'NONE',  ( -13.34999999999999076, 2.500000000000000000, 1.372243186433549367 ) ) ;
#85353=ORIENTED_EDGE ( 'NONE', *, *, #31418, .T. ) ;
#85354=ORIENTED_EDGE ( 'NONE', *, *, #55480, .F. ) ;
#85355=ORIENTED_EDGE ( 'NONE', *, *, #98914, .F. ) ;
#85356=ORIENTED_EDGE ( 'NONE', *, *, #72157, .T. ) ;
#85357=DIRECTION ( 'NONE',  ( 0.000000000000000000, 1.000000000000000000, 0.000000000000000000 ) ) ;
#85358=ORIENTED_EDGE ( 'NONE', *, *, #119914, .T. ) ;
#85359=CIRCLE ( 'NONE', #8079, 0.06509327318403745899 ) ;
#85360=FACE_OUTER_BOUND ( 'NONE', #85639, .T. ) ;
#85361=ORIENTED_EDGE ( 'NONE', *, *, #68774, .F. ) ;
#85362=ORIENTED_EDGE ( 'NONE', *, *, #30343, .T. ) ;
#85364=VECTOR ( 'NONE', #95579, 1000.000000000000000 ) ;
#85365=AXIS2_PLACEMENT_3D ( 'NONE', #64466, #4244, #23917 ) ;
#85366=CARTESIAN_POINT ( 'NONE',  ( -0.8500000000000386136, 2.500000000000000000, 5.902370205355745192 ) ) ;
#85367=CIRCLE ( 'NONE', #20538, 0.06509327318403745899 ) ;
#85368=CARTESIAN_POINT ( 'NONE',  ( 9.599999999999917932, 12.50000000000000000, 0.6928203230275494784 ) ) ;
#85369=CARTESIAN_POINT ( 'NONE',  ( 12.49999999999993960, 2.500000000000000000, -4.230127018922201998 ) ) ;
#85370=ORIENTED_EDGE ( 'NONE', *, *, #3434, .T. ) ;
#85371=CIRCLE ( 'NONE', #28955, 0.1000000000000000056 ) ;
#85372=CIRCLE ( 'NONE', #93793, 0.06509327318403741736 ) ;
#85373=ORIENTED_EDGE ( 'NONE', *, *, #73494, .F. ) ;
#85374=ADVANCED_FACE ( 'NONE', ( #107281 ), #118388, .T. ) ;
#85375=CIRCLE ( 'NONE', #41495, 0.1000000000000002554 ) ;
#85376=EDGE_LOOP ( 'NONE', ( #71930, #121320 ) ) ;
#85377=DIRECTION ( 'NONE',  ( 0.000000000000000000, 0.000000000000000000, 1.000000000000000000 ) ) ;
#85378=EDGE_LOOP ( 'NONE', ( #22773, #101718 ) ) ;
#85380=CARTESIAN_POINT ( 'NONE',  ( 13.34999999999990017, 2.500000000000000000, 2.957883832488649389 ) ) ;
#85381=EDGE_LOOP ( 'NONE', ( #129154, #82342, #18729, #83577 ) ) ;
#85382=ORIENTED_EDGE ( 'NONE', *, *, #87733, .T. ) ;
#85383=AXIS2_PLACEMENT_3D ( 'NONE', #118305, #98013, #109109 ) ;
#85385=EDGE_CURVE ( 'NONE', #29210, #112782, #108442, .T. ) ;
#85386=CIRCLE ( 'NONE', #74927, 0.06509327318403745899 ) ;
#85387=CARTESIAN_POINT ( 'NONE',  ( -13.74999999999998757, 2.500000000000000000, -2.957883832488651610 ) ) ;
#85388=DIRECTION ( 'NONE',  ( -0.000000000000000000, -1.000000000000000000, -0.000000000000000000 ) ) ;
#85390=DIRECTION ( 'NONE',  ( 0.000000000000000000, -0.000000000000000000, 1.000000000000000000 ) ) ;
#85391=CARTESIAN_POINT ( 'NONE',  ( 7.099999999999928590, 2.500000000000000000, 4.330127018922196314 ) ) ;
#85392=EDGE_LOOP ( 'NONE', ( #92455, #28149 ) ) ;
#85393=FACE_OUTER_BOUND ( 'NONE', #94867, .T. ) ;
#85394=CIRCLE ( 'NONE', #41511, 0.1000000000000002554 ) ;
#85395=VERTEX_POINT ( 'NONE', #119045 ) ;
#85396=CARTESIAN_POINT ( 'NONE',  ( 7.899999999999923084, 2.500000000000000000, 0.6928203230275494784 ) ) ;
#85397=ORIENTED_EDGE ( 'NONE', *, *, #30711, .T. ) ;
#85398=PLANE ( 'NONE',  #84949 ) ;
#85399=PLANE ( 'NONE',  #53262 ) ;
#85400=AXIS2_PLACEMENT_3D ( 'NONE', #126571, #29025, #68926 ) ;
#85401=AXIS2_PLACEMENT_3D ( 'NONE', #6658, #96349, #127760 ) ;
#85402=EDGE_LOOP ( 'NONE', ( #155, #16, #1308, #13250 ) ) ;
#85403=DIRECTION ( 'NONE',  ( 0.000000000000000000, 0.000000000000000000, 1.000000000000000000 ) ) ;
#85404=DIRECTION ( 'NONE',  ( 0.000000000000000000, 0.000000000000000000, 1.000000000000000000 ) ) ;
#85405=ORIENTED_EDGE ( 'NONE', *, *, #57837, .T. ) ;
#85406=CARTESIAN_POINT ( 'NONE',  ( 2.899999999999943956, 12.50000000000000000, 4.395220292106234439 ) ) ;
#85407=VECTOR ( 'NONE', #18273, 1000.000000000000000 ) ;
#85408=DIRECTION ( 'NONE',  ( 0.000000000000000000, 0.000000000000000000, 1.000000000000000000 ) ) ;
#85409=EDGE_LOOP ( 'NONE', ( #51773, #26253 ) ) ;
#85410=ORIENTED_EDGE ( 'NONE', *, *, #56479, .T. ) ;
#85411=DIRECTION ( 'NONE',  ( -0.000000000000000000, 1.000000000000000000, -0.000000000000000000 ) ) ;
#85412=CARTESIAN_POINT ( 'NONE',  ( -12.09999999999999432, 2.500000000000000000, 5.022947341949748790 ) ) ;
#85414=DIRECTION ( 'NONE',  ( -0.000000000000000000, 1.000000000000000000, -0.000000000000000000 ) ) ;
#85415=VECTOR ( 'NONE', #1027, 1000.000000000000000 ) ;
#85416=EDGE_CURVE ( 'NONE', #15482, #84687, #96166, .T. ) ;
#85417=AXIS2_PLACEMENT_3D ( 'NONE', #27017, #79347, #108141 ) ;
#85418=CARTESIAN_POINT ( 'NONE',  ( 13.09999999999990195, 12.50000000000000000, -4.741630453620016006 ) ) ;
#85419=DIRECTION ( 'NONE',  ( 0.000000000000000000, 0.000000000000000000, -1.000000000000000000 ) ) ;
#85420=AXIS2_PLACEMENT_3D ( 'NONE', #103553, #83888, #74080 ) ;
#85421=VERTEX_POINT ( 'NONE', #26792 ) ;
#85422=CARTESIAN_POINT ( 'NONE',  ( 26.76179944288227475, 1.073660921396622614, -4.445808334545023222 ) ) ;
#85423=ORIENTED_EDGE ( 'NONE', *, *, #23125, .T. ) ;
#85424=AXIS2_PLACEMENT_3D ( 'NONE', #69352, #41857, #101414 ) ;
#85425=EDGE_CURVE ( 'NONE', #12748, #90660, #89674, .T. ) ;
#85426=CONICAL_SURFACE ( 'NONE', #106356, 0.1000000000000002554, 0.003490658503988666988 ) ;
#85427=DIRECTION ( 'NONE',  ( 0.000000000000000000, 0.000000000000000000, 1.000000000000000000 ) ) ;
#85428=DIRECTION ( 'NONE',  ( 0.000000000000000000, -0.9999939076577903929, 0.003490651415223739937 ) ) ;
#85429=EDGE_CURVE ( 'NONE', #118375, #88991, #52241, .T. ) ;
#85430=DIRECTION ( 'NONE',  ( -0.000000000000000000, 1.000000000000000000, -0.000000000000000000 ) ) ;
#85431=VERTEX_POINT ( 'NONE', #92149 ) ;
#85432=CIRCLE ( 'NONE', #58260, 0.1000000000000002554 ) ;
#85433=CIRCLE ( 'NONE', #6002, 0.06509327318403745899 ) ;
#85434=DIRECTION ( 'NONE',  ( 0.000000000000000000, 0.000000000000000000, 1.000000000000000000 ) ) ;
#85435=DIRECTION ( 'NONE',  ( 0.000000000000000000, -0.000000000000000000, 1.000000000000000000 ) ) ;
#85436=EDGE_CURVE ( 'NONE', #116432, #22907, #60769, .T. ) ;
#85437=EDGE_LOOP ( 'NONE', ( #6027, #75369, #17532, #33349 ) ) ;
#85438=CARTESIAN_POINT ( 'NONE',  ( 3.749999999999976907, 2.500000000000000000, 2.165063509461097713 ) ) ;
#85439=EDGE_LOOP ( 'NONE', ( #11755, #38574, #38681, #41277 ) ) ;
#85440=ORIENTED_EDGE ( 'NONE', *, *, #100239, .T. ) ;
#85441=CARTESIAN_POINT ( 'NONE',  ( -2.500000000000032863, 2.500000000000000000, 5.022947341949748790 ) ) ;
#85443=ORIENTED_EDGE ( 'NONE', *, *, #8951, .T. ) ;
#85444=DIRECTION ( 'NONE',  ( 0.000000000000000000, -0.9999939076577903929, 0.003490651415223739937 ) ) ;
#85445=CARTESIAN_POINT ( 'NONE',  ( -12.49999999999995737, 2.500000000000000000, 4.330127018922196314 ) ) ;
#85446=DIRECTION ( 'NONE',  ( 0.000000000000000000, 0.000000000000000000, 1.000000000000000000 ) ) ;
#85447=ORIENTED_EDGE ( 'NONE', *, *, #101532, .T. ) ;
#85448=AXIS2_PLACEMENT_3D ( 'NONE', #37943, #107972, #20239 ) ;
#85449=FACE_BOUND ( 'NONE', #116713, .T. ) ;
#85450=AXIS2_PLACEMENT_3D ( 'NONE', #86024, #51304, #80754 ) ;
#85451=AXIS2_PLACEMENT_3D ( 'NONE', #43715, #52869, #2453 ) ;
#85452=CARTESIAN_POINT ( 'NONE',  ( -6.700000000000019718, 2.500000000000000000, -4.330127018922201643 ) ) ;
#85453=ORIENTED_EDGE ( 'NONE', *, *, #90171, .F. ) ;
#85454=DIRECTION ( 'NONE',  ( 0.000000000000000000, -0.000000000000000000, 1.000000000000000000 ) ) ;
#85455=DIRECTION ( 'NONE',  ( 0.000000000000000000, 0.000000000000000000, 1.000000000000000000 ) ) ;
#85456=AXIS2_PLACEMENT_3D ( 'NONE', #83502, #33739, #86707 ) ;
#85457=ORIENTED_EDGE ( 'NONE', *, *, #115973, .T. ) ;
#85458=CIRCLE ( 'NONE', #79221, 0.1000000000000000472 ) ;
#85459=ADVANCED_FACE ( 'NONE', ( #69943 ), #90201, .T. ) ;
#85460=CONICAL_SURFACE ( 'NONE', #43729, 0.1000000000000002554, 0.003490658503988666988 ) ;
#85461=VERTEX_POINT ( 'NONE', #120334 ) ;
#85462=ORIENTED_EDGE ( 'NONE', *, *, #81361, .F. ) ;
#85463=LINE ( 'NONE', #75010, #60810 ) ;
#85464=CARTESIAN_POINT ( 'NONE',  ( 2.500000000000002220, 1.499999999999999556, 10.00000000000000533 ) ) ;
#85465=CARTESIAN_POINT ( 'NONE',  ( -10.65000000000000213, 2.500000000000000000, 1.718653347947321386 ) ) ;
#85466=ADVANCED_FACE ( 'NONE', ( #2465 ), #16490, .T. ) ;
#85467=FACE_BOUND ( 'NONE', #115580, .T. ) ;
#85468=ORIENTED_EDGE ( 'NONE', *, *, #20282, .T. ) ;
#85470=VECTOR ( 'NONE', #124099, 1000.000000000000000 ) ;
#85471=EDGE_CURVE ( 'NONE', #60027, #91650, #52030, .T. ) ;
#85472=CARTESIAN_POINT ( 'NONE',  ( -10.85000000000000142, 2.500000000000000000, 6.395190528383296602 ) ) ;
#85473=DIRECTION ( 'NONE',  ( 0.000000000000000000, -0.000000000000000000, 1.000000000000000000 ) ) ;
#85474=CONICAL_SURFACE ( 'NONE', #33274, 0.1000000000000002554, 0.003490658503988666988 ) ;
#85476=ADVANCED_FACE ( 'NONE', ( #101341 ), #110504, .T. ) ;
#85477=CARTESIAN_POINT ( 'NONE',  ( 0.6499999999999543920, 12.50000000000000000, 6.841600689897072485 ) ) ;
#85478=ADVANCED_FACE ( 'NONE', ( #1832 ), #122274, .T. ) ;
#85479=CARTESIAN_POINT ( 'NONE',  ( -9.999999999999969802, 12.50000000000000000, 4.330127018922196314 ) ) ;
#85480=EDGE_CURVE ( 'NONE', #9421, #55696, #123124, .T. ) ;
#85481=DIRECTION ( 'NONE',  ( 0.000000000000000000, -0.000000000000000000, 1.000000000000000000 ) ) ;
#85482=CARTESIAN_POINT ( 'NONE',  ( 1.049999999999953637, 12.50000000000000000, 2.446380397790835826 ) ) ;
#85483=CIRCLE ( 'NONE', #70811, 0.06509327318403745899 ) ;
#85484=DIRECTION ( 'NONE',  ( 0.000000000000000000, 1.000000000000000000, 0.000000000000000000 ) ) ;
#85485=ADVANCED_FACE ( 'NONE', ( #109204 ), #66670, .T. ) ;
#85486=EDGE_LOOP ( 'NONE', ( #46105, #12742 ) ) ;
#85487=ORIENTED_EDGE ( 'NONE', *, *, #37254, .F. ) ;
#85488=ORIENTED_EDGE ( 'NONE', *, *, #35223, .F. ) ;
#85489=ORIENTED_EDGE ( 'NONE', *, *, #1260, .F. ) ;
#85490=ORIENTED_EDGE ( 'NONE', *, *, #67434, .T. ) ;
#85491=AXIS2_PLACEMENT_3D ( 'NONE', #89766, #93, #7003 ) ;
#85492=FACE_OUTER_BOUND ( 'NONE', #8445, .T. ) ;
#85493=DIRECTION ( 'NONE',  ( 0.000000000000000000, 0.000000000000000000, -1.000000000000000000 ) ) ;
#85494=EDGE_LOOP ( 'NONE', ( #105237, #48865 ) ) ;
#85495=FACE_BOUND ( 'NONE', #123349, .T. ) ;
#85496=EDGE_CURVE ( 'NONE', #76941, #82898, #10253, .T. ) ;
#85497=DIRECTION ( 'NONE',  ( 0.000000000000000000, 1.000000000000000000, 0.000000000000000000 ) ) ;
#85498=AXIS2_PLACEMENT_3D ( 'NONE', #72390, #112941, #41007 ) ;
#85499=CARTESIAN_POINT ( 'NONE',  ( -9.150000000000009237, 12.50000000000000000, -7.188010851410848723 ) ) ;
#85500=ORIENTED_EDGE ( 'NONE', *, *, #71387, .T. ) ;
#85501=DIRECTION ( 'NONE',  ( -0.000000000000000000, 1.000000000000000000, -0.000000000000000000 ) ) ;
#85502=CARTESIAN_POINT ( 'NONE',  ( 2.699999999999947331, 12.50000000000000000, -0.3464101615137783474 ) ) ;
#85503=CARTESIAN_POINT ( 'NONE',  ( -8.750000000000010658, 12.50000000000000000, -7.188010851410848723 ) ) ;
#85504=ORIENTED_EDGE ( 'NONE', *, *, #98313, .T. ) ;
#85505=DIRECTION ( 'NONE',  ( 0.000000000000000000, 1.000000000000000000, 0.000000000000000000 ) ) ;
#85506=AXIS2_PLACEMENT_3D ( 'NONE', #88326, #28797, #18947 ) ;
#85507=VERTEX_POINT ( 'NONE', #89580 ) ;
#85508=ORIENTED_EDGE ( 'NONE', *, *, #71396, .F. ) ;
#85509=EDGE_LOOP ( 'NONE', ( #91835, #79292, #41917, #30587 ) ) ;
#85510=CARTESIAN_POINT ( 'NONE',  ( -2.950000000000030376, 12.50000000000000000, 6.560283801567334372 ) ) ;
#85511=DIRECTION ( 'NONE',  ( 0.000000000000000000, 0.000000000000000000, 1.000000000000000000 ) ) ;
#85512=FACE_OUTER_BOUND ( 'NONE', #13392, .T. ) ;
#85513=VECTOR ( 'NONE', #114190, 1000.000000000000000 ) ;
#85514=VERTEX_POINT ( 'NONE', #10374 ) ;
#85515=CARTESIAN_POINT ( 'NONE',  ( 14.38463633427375576, 1.500000000000064171, -7.683002070836549180 ) ) ;
#85516=CARTESIAN_POINT ( 'NONE',  ( -8.100000000000010303, 2.500000000000000000, 4.676537180435972552 ) ) ;
#85517=AXIS2_PLACEMENT_3D ( 'NONE', #93005, #3960, #42627 ) ;
#85518=FACE_OUTER_BOUND ( 'NONE', #128559, .T. ) ;
#85519=AXIS2_PLACEMENT_3D ( 'NONE', #55538, #73238, #123607 ) ;
#85521=DIRECTION ( 'NONE',  ( 0.000000000000000000, 0.000000000000000000, 1.000000000000000000 ) ) ;
#85522=CIRCLE ( 'NONE', #45824, 0.1000000000000002554 ) ;
#85523=PLANE ( 'NONE',  #68353 ) ;
#85524=ORIENTED_EDGE ( 'NONE', *, *, #114808, .F. ) ;
#85525=CARTESIAN_POINT ( 'NONE',  ( 1.449999999999951328, 12.50000000000000000, 2.446380397790835826 ) ) ;
#85526=CIRCLE ( 'NONE', #62561, 0.1000000000000002554 ) ;
#85527=AXIS2_PLACEMENT_3D ( 'NONE', #68536, #1724, #119564 ) ;
#85528=VERTEX_POINT ( 'NONE', #1196 ) ;
#85529=EDGE_CURVE ( 'NONE', #81382, #26297, #68737, .T. ) ;
#85530=ORIENTED_EDGE ( 'NONE', *, *, #24573, .F. ) ;
#85531=FACE_OUTER_BOUND ( 'NONE', #64372, .T. ) ;
#85532=CARTESIAN_POINT ( 'NONE',  ( -4.200000000000029488, 2.500000000000000000, -4.330127018922201643 ) ) ;
#85533=DIRECTION ( 'NONE',  ( -4.274815082592931898E-19, -0.9999939076577903929, -0.003490651415223739937 ) ) ;
#85534=ORIENTED_EDGE ( 'NONE', *, *, #66760, .T. ) ;
#85535=VERTEX_POINT ( 'NONE', #99414 ) ;
#85536=EDGE_CURVE ( 'NONE', #107774, #118072, #104251, .T. ) ;
#85537=DIRECTION ( 'NONE',  ( 0.000000000000000000, 0.000000000000000000, 1.000000000000000000 ) ) ;
#85538=DIRECTION ( 'NONE',  ( 0.000000000000000000, 0.000000000000000000, -1.000000000000000000 ) ) ;
#85539=DIRECTION ( 'NONE',  ( -0.000000000000000000, -1.000000000000000000, -0.000000000000000000 ) ) ;
#85540=CONICAL_SURFACE ( 'NONE', #31271, 0.1000000000000002554, 0.003490658503988666988 ) ;
#85541=EDGE_LOOP ( 'NONE', ( #93566, #48316 ) ) ;
#85542=EDGE_LOOP ( 'NONE', ( #74480, #128774 ) ) ;
#85543=DIRECTION ( 'NONE',  ( 0.000000000000000000, 0.000000000000000000, 1.000000000000000000 ) ) ;
#85545=CARTESIAN_POINT ( 'NONE',  ( -8.100000000000010303, 12.50000000000000000, 4.676537180435972552 ) ) ;
#85546=VECTOR ( 'NONE', #82375, 1000.000000000000000 ) ;
#85547=PLANE ( 'NONE',  #67920 ) ;
#85548=ORIENTED_EDGE ( 'NONE', *, *, #76389, .T. ) ;
#85549=DIRECTION ( 'NONE',  ( 0.000000000000000000, 0.000000000000000000, 1.000000000000000000 ) ) ;
#85550=LINE ( 'NONE', #63341, #104797 ) ;
#85551=CARTESIAN_POINT ( 'NONE',  ( -9.350000000000006750, 2.500000000000000000, -2.411473670974877859 ) ) ;
#85552=DIRECTION ( 'NONE',  ( -0.000000000000000000, 1.000000000000000000, -0.000000000000000000 ) ) ;
#85553=AXIS2_PLACEMENT_3D ( 'NONE', #102336, #2838, #42797 ) ;
#85554=ORIENTED_EDGE ( 'NONE', *, *, #73250, .F. ) ;
#85555=AXIS2_PLACEMENT_3D ( 'NONE', #104553, #114365, #73167 ) ;
#85556=VECTOR ( 'NONE', #93590, 1000.000000000000000 ) ;
#85557=DIRECTION ( 'NONE',  ( 0.000000000000000000, 0.000000000000000000, 1.000000000000000000 ) ) ;
#85559=VERTEX_POINT ( 'NONE', #49677 ) ;
#85560=ORIENTED_EDGE ( 'NONE', *, *, #52533, .T. ) ;
#85561=CARTESIAN_POINT ( 'NONE',  ( -0.8500000000000395017, 2.500000000000000000, 6.595190528383296780 ) ) ;
#85562=DIRECTION ( 'NONE',  ( 0.000000000000000000, 0.000000000000000000, -1.000000000000000000 ) ) ;
#85563=DIRECTION ( 'NONE',  ( 0.000000000000000000, 1.000000000000000000, 0.000000000000000000 ) ) ;
#85564=DIRECTION ( 'NONE',  ( 0.000000000000000000, 0.000000000000000000, -1.000000000000000000 ) ) ;
#85565=CONICAL_SURFACE ( 'NONE', #26998, 0.09999999999999982514, 0.003490658503988666988 ) ;
#85566=CARTESIAN_POINT ( 'NONE',  ( 4.599999999999936584, 2.500000000000000000, 3.737306695894644371 ) ) ;
#85567=CARTESIAN_POINT ( 'NONE',  ( 9.999999999999916511, 2.500000000000000000, -0.6928203230275541413 ) ) ;
#85568=AXIS2_PLACEMENT_3D ( 'NONE', #40868, #38939, #80780 ) ;
#85569=ADVANCED_FACE ( 'NONE', ( #111125 ), #77151, .T. ) ;
#85570=AXIS2_PLACEMENT_3D ( 'NONE', #57781, #39451, #97687 ) ;
#85571=DIRECTION ( 'NONE',  ( 0.000000000000000000, 0.000000000000000000, 1.000000000000000000 ) ) ;
#85572=CARTESIAN_POINT ( 'NONE',  ( -1.050000000000038680, 2.500000000000000000, 6.941600689897073018 ) ) ;
#85574=DIRECTION ( 'NONE',  ( -0.000000000000000000, 1.000000000000000000, -0.000000000000000000 ) ) ;
#85575=CARTESIAN_POINT ( 'NONE',  ( -1.650000000000034328, 12.50000000000000000, -2.099970236277064473 ) ) ;
#85576=EDGE_CURVE ( 'NONE', #30501, #54077, #47828, .T. ) ;
#85577=VERTEX_POINT ( 'NONE', #538 ) ;
#85579=AXIS2_PLACEMENT_3D ( 'NONE', #119540, #107802, #29888 ) ;
#85580=EDGE_CURVE ( 'NONE', #115716, #33086, #40506, .T. ) ;
#85581=ORIENTED_EDGE ( 'NONE', *, *, #112053, .F. ) ;
#85582=DIRECTION ( 'NONE',  ( 0.000000000000000000, 0.000000000000000000, 1.000000000000000000 ) ) ;
#85583=EDGE_CURVE ( 'NONE', #117286, #54541, #22795, .T. ) ;
#85584=LINE ( 'NONE', #107146, #23390 ) ;
#85586=CARTESIAN_POINT ( 'NONE',  ( 21.23528140090950700, -2.699413673072311948, -2.293764360948876480 ) ) ;
#85587=ADVANCED_FACE ( 'NONE', ( #65251 ), #98071, .T. ) ;
#85588=DIRECTION ( 'NONE',  ( 0.000000000000000000, 0.000000000000000000, -1.000000000000000000 ) ) ;
#85589=DIRECTION ( 'NONE',  ( 0.000000000000000000, 0.000000000000000000, 1.000000000000000000 ) ) ;
#85591=EDGE_CURVE ( 'NONE', #95448, #98294, #47920, .T. ) ;
#85592=CIRCLE ( 'NONE', #89708, 0.06509327318403745899 ) ;
#85593=CARTESIAN_POINT ( 'NONE',  ( -2.050000000000032685, 12.50000000000000000, -2.165063509461101710 ) ) ;
#85594=ORIENTED_EDGE ( 'NONE', *, *, #81033, .T. ) ;
#85595=ORIENTED_EDGE ( 'NONE', *, *, #115306, .F. ) ;
#85597=VERTEX_POINT ( 'NONE', #43087 ) ;
#85598=DIRECTION ( 'NONE',  ( 0.000000000000000000, 0.000000000000000000, 1.000000000000000000 ) ) ;
#85599=AXIS2_PLACEMENT_3D ( 'NONE', #2139, #109529, #91172 ) ;
#85600=CARTESIAN_POINT ( 'NONE',  ( 8.349999999999919709, 2.500000000000000000, 5.702370205355745014 ) ) ;
#85601=CARTESIAN_POINT ( 'NONE',  ( -12.09999999999999609, 2.500000000000000000, 0.6928203230275535862 ) ) ;
#85602=DIRECTION ( 'NONE',  ( 0.000000000000000000, 0.000000000000000000, 1.000000000000000000 ) ) ;
#85603=VERTEX_POINT ( 'NONE', #24711 ) ;
#85604=AXIS2_PLACEMENT_3D ( 'NONE', #37145, #106513, #97978 ) ;
#85605=AXIS2_PLACEMENT_3D ( 'NONE', #111717, #79674, #121515 ) ;
#85606=CARTESIAN_POINT ( 'NONE',  ( -4.600000000000028066, 12.50000000000000000, -5.022947341949754119 ) ) ;
#85607=ORIENTED_EDGE ( 'NONE', *, *, #67271, .T. ) ;
#85608=DIRECTION ( 'NONE',  ( 0.000000000000000000, -0.9999939076577903929, 0.003490651415223739937 ) ) ;
#85609=CARTESIAN_POINT ( 'NONE',  ( 14.69205215096692818, -2.499999999999999112, -6.336420066640019222 ) ) ;
#85610=CIRCLE ( 'NONE', #31253, 0.1000000000000000472 ) ;
#85611=DIRECTION ( 'NONE',  ( 0.000000000000000000, 0.000000000000000000, 1.000000000000000000 ) ) ;
#85612=CARTESIAN_POINT ( 'NONE',  ( 15.86953761860680068, -2.463355995079608451, 3.896699429476443211 ) ) ;
#85613=ORIENTED_EDGE ( 'NONE', *, *, #30809, .T. ) ;
#85614=VECTOR ( 'NONE', #16154, 1000.000000000000000 ) ;
#85615=AXIS2_PLACEMENT_3D ( 'NONE', #5582, #57286, #77554 ) ;
#85616=EDGE_CURVE ( 'NONE', #54196, #106953, #31199, .T. ) ;
#85618=EDGE_LOOP ( 'NONE', ( #79889, #21626, #118031, #108476 ) ) ;
#85619=LINE ( 'NONE', #125540, #33544 ) ;
#85620=CARTESIAN_POINT ( 'NONE',  ( -2.100000000000034284, 2.500000000000000000, -4.330127018922201643 ) ) ;
#85621=CARTESIAN_POINT ( 'NONE',  ( -1.700000000000034817, 2.500000000000000000, -0.1000000000000023925 ) ) ;
#85622=FACE_BOUND ( 'NONE', #16174, .T. ) ;
#85623=CARTESIAN_POINT ( 'NONE',  ( 4.199999999999938005, 2.500000000000000000, 4.430127018922196847 ) ) ;
#85624=CARTESIAN_POINT ( 'NONE',  ( 6.249999999999930722, 12.50000000000000000, 1.472243186433545459 ) ) ;
#85625=EDGE_CURVE ( 'NONE', #11699, #32199, #50075, .T. ) ;
#85626=CARTESIAN_POINT ( 'NONE',  ( 12.69999999999990159, 2.500000000000000000, 4.776537180435972196 ) ) ;
#85627=DIRECTION ( 'NONE',  ( 0.000000000000000000, 0.000000000000000000, 1.000000000000000000 ) ) ;
#85628=VECTOR ( 'NONE', #118661, 1000.000000000000000 ) ;
#85629=EDGE_CURVE ( 'NONE', #8254, #30750, #27074, .T. ) ;
#85631=LINE ( 'NONE', #106554, #92646 ) ;
#85632=EDGE_CURVE ( 'NONE', #28676, #121748, #125270, .T. ) ;
#85633=DIRECTION ( 'NONE',  ( 0.000000000000000000, 1.000000000000000000, 0.000000000000000000 ) ) ;
#85634=ADVANCED_FACE ( 'NONE', ( #82998 ), #62710, .T. ) ;
#85635=VECTOR ( 'NONE', #119830, 1000.000000000000000 ) ;
#85636=VECTOR ( 'NONE', #104571, 1000.000000000000000 ) ;
#85637=CARTESIAN_POINT ( 'NONE',  ( 2.099999999999948574, 12.50000000000000000, 3.637306695894644726 ) ) ;
#85638=ADVANCED_FACE ( 'NONE', ( #43725 ), #104341, .T. ) ;
#85639=EDGE_LOOP ( 'NONE', ( #110105, #28039, #122308, #7740 ) ) ;
#85640=EDGE_LOOP ( 'NONE', ( #106560, #122092, #82892, #115272 ) ) ;
#85641=ORIENTED_EDGE ( 'NONE', *, *, #98895, .F. ) ;
#85642=EDGE_LOOP ( 'NONE', ( #13645, #20180, #12115, #11789 ) ) ;
#85643=DIRECTION ( 'NONE',  ( 0.000000000000000000, 1.000000000000000000, 0.000000000000000000 ) ) ;
#85644=FACE_BOUND ( 'NONE', #81039, .T. ) ;
#85645=DIRECTION ( 'NONE',  ( 0.000000000000000000, 0.000000000000000000, 1.000000000000000000 ) ) ;
#85646=AXIS2_PLACEMENT_3D ( 'NONE', #34084, #32163, #71404 ) ;
#85647=VECTOR ( 'NONE', #25843, 1000.000000000000000 ) ;
#85648=CIRCLE ( 'NONE', #43901, 0.06509327318403745899 ) ;
#85649=EDGE_CURVE ( 'NONE', #33086, #109058, #129504, .T. ) ;
#85651=ORIENTED_EDGE ( 'NONE', *, *, #99515, .T. ) ;
#85652=CARTESIAN_POINT ( 'NONE',  ( 3.149999999999946176, 2.500000000000000000, -2.411473670974877859 ) ) ;
#85653=CARTESIAN_POINT ( 'NONE',  ( -0.6500000000000398792, 2.500000000000000000, -6.941600689897078347 ) ) ;
#85654=VERTEX_POINT ( 'NONE', #73794 ) ;
#85655=DIRECTION ( 'NONE',  ( 0.000000000000000000, 1.000000000000000000, 0.000000000000000000 ) ) ;
#85656=CARTESIAN_POINT ( 'NONE',  ( 9.799999999999913669, 12.50000000000000000, 4.741630453620009789 ) ) ;
#85657=AXIS2_PLACEMENT_3D ( 'NONE', #77389, #45365, #27005 ) ;
#85658=AXIS2_PLACEMENT_3D ( 'NONE', #91740, #11231, #81283 ) ;
#85659=EDGE_LOOP ( 'NONE', ( #115244, #77342, #13064, #65066 ) ) ;
#85660=CARTESIAN_POINT ( 'NONE',  ( 6.699999999999930012, 2.500000000000000000, 4.230127018922196669 ) ) ;
#85661=DIRECTION ( 'NONE',  ( 0.000000000000000000, 0.000000000000000000, 1.000000000000000000 ) ) ;
#85663=ORIENTED_EDGE ( 'NONE', *, *, #20081, .F. ) ;
#85664=PLANE ( 'NONE',  #103247 ) ;
#85665=CARTESIAN_POINT ( 'NONE',  ( 13.74999999999993427, 2.500000000000000000, 2.165063509461097713 ) ) ;
#85666=EDGE_LOOP ( 'NONE', ( #85595, #84771, #14128, #36757 ) ) ;
#85667=FACE_OUTER_BOUND ( 'NONE', #113765, .T. ) ;
#85668=CIRCLE ( 'NONE', #119126, 0.1000000000000000472 ) ;
#85669=ORIENTED_EDGE ( 'NONE', *, *, #124056, .F. ) ;
#85670=ORIENTED_EDGE ( 'NONE', *, *, #80465, .T. ) ;
#85671=CARTESIAN_POINT ( 'NONE',  ( 10.84999999999990905, 12.50000000000000000, 1.472243186433545459 ) ) ;
#85672=VERTEX_POINT ( 'NONE', #102611 ) ;
#85673=DIRECTION ( 'NONE',  ( 0.000000000000000000, 0.000000000000000000, 1.000000000000000000 ) ) ;
#85674=CARTESIAN_POINT ( 'NONE',  ( -10.65000000000000213, 2.500000000000000000, 6.741600689897071952 ) ) ;
#85675=VERTEX_POINT ( 'NONE', #74452 ) ;
#85676=DIRECTION ( 'NONE',  ( -0.000000000000000000, 1.000000000000000000, -0.000000000000000000 ) ) ;
#85677=DIRECTION ( 'NONE',  ( -0.000000000000000000, 1.000000000000000000, -0.000000000000000000 ) ) ;
#85678=CARTESIAN_POINT ( 'NONE',  ( -1.050000000000037792, 12.50000000000000000, 1.818653347947321475 ) ) ;
#85679=CARTESIAN_POINT ( 'NONE',  ( 1.249999999999952038, 12.50000000000000000, 5.737276932171707422 ) ) ;
#85680=CARTESIAN_POINT ( 'NONE',  ( -11.24999999999996270, 2.500000000000000000, 6.595190528383296780 ) ) ;
#85681=CARTESIAN_POINT ( 'NONE',  ( 17.50011966276722220, 2.224296756944650344, -4.070989939659154011 ) ) ;
#85682=ORIENTED_EDGE ( 'NONE', *, *, #87652, .T. ) ;
#85683=ADVANCED_FACE ( 'NONE', ( #52881 ), #55454, .T. ) ;
#85684=VERTEX_POINT ( 'NONE', #53532 ) ;
#85685=DIRECTION ( 'NONE',  ( 0.000000000000000000, 0.000000000000000000, 1.000000000000000000 ) ) ;
#85686=CARTESIAN_POINT ( 'NONE',  ( 16.55874544816229132, -0.4845305829427751232, 6.091953208798936537 ) ) ;
#85687=CARTESIAN_POINT ( 'NONE',  ( 13.14999999999989733, 2.500000000000000000, -1.818653347947325916 ) ) ;
#85688=ORIENTED_EDGE ( 'NONE', *, *, #63493, .T. ) ;
#85689=ORIENTED_EDGE ( 'NONE', *, *, #68880, .F. ) ;
#85690=ORIENTED_EDGE ( 'NONE', *, *, #66007, .F. ) ;
#85691=AXIS2_PLACEMENT_3D ( 'NONE', #69927, #7769, #58189 ) ;
#85692=DIRECTION ( 'NONE',  ( 0.000000000000000000, 0.000000000000000000, 1.000000000000000000 ) ) ;
#85693=CARTESIAN_POINT ( 'NONE',  ( -8.100000000000013856, 2.500000000000000000, 0.2464101615137736789 ) ) ;
#85696=CIRCLE ( 'NONE', #102434, 0.06509327318403745899 ) ;
#85697=CIRCLE ( 'NONE', #20864, 0.1000000000000002554 ) ;
#85698=DIRECTION ( 'NONE',  ( -0.000000000000000000, -1.000000000000000000, -0.000000000000000000 ) ) ;
#85699=CARTESIAN_POINT ( 'NONE',  ( 7.049999999999928768, 12.50000000000000000, 6.560283801567334372 ) ) ;
#85700=DIRECTION ( 'NONE',  ( -0.000000000000000000, 1.000000000000000000, -0.000000000000000000 ) ) ;
#85701=DIRECTION ( 'NONE',  ( 0.000000000000000000, 1.000000000000000000, 0.000000000000000000 ) ) ;
#85702=DIRECTION ( 'NONE',  ( 0.000000000000000000, 1.000000000000000000, 0.000000000000000000 ) ) ;
#85703=PLANE ( 'NONE',  #28956 ) ;
#85704=VECTOR ( 'NONE', #82030, 1000.000000000000000 ) ;
#85705=AXIS2_PLACEMENT_3D ( 'NONE', #77882, #126356, #128301 ) ;
#85706=ORIENTED_EDGE ( 'NONE', *, *, #61415, .T. ) ;
#85707=DIRECTION ( 'NONE',  ( 0.000000000000000000, 1.000000000000000000, 0.000000000000000000 ) ) ;
#85708=ORIENTED_EDGE ( 'NONE', *, *, #64896, .T. ) ;
#85709=ORIENTED_EDGE ( 'NONE', *, *, #101403, .T. ) ;
#85710=PLANE ( 'NONE',  #60927 ) ;
#85711=DIRECTION ( 'NONE',  ( 0.000000000000000000, -0.000000000000000000, 1.000000000000000000 ) ) ;
#85712=DIRECTION ( 'NONE',  ( 0.000000000000000000, 0.000000000000000000, -1.000000000000000000 ) ) ;
#85713=CARTESIAN_POINT ( 'NONE',  ( 4.599999999999938360, 2.500000000000000000, 0.09999999999999772959 ) ) ;
#85714=DIRECTION ( 'NONE',  ( 0.000000000000000000, 1.000000000000000000, 0.000000000000000000 ) ) ;
#85715=CARTESIAN_POINT ( 'NONE',  ( 1.049999999999953637, 2.500000000000000000, 2.511473670974873507 ) ) ;
#85716=LINE ( 'NONE', #67338, #99158 ) ;
#85717=ORIENTED_EDGE ( 'NONE', *, *, #116327, .T. ) ;
#85718=PLANE ( 'NONE',  #59860 ) ;
#85719=CARTESIAN_POINT ( 'NONE',  ( 5.849999999999933920, 2.500000000000000000, -2.165063509461101710 ) ) ;
#85720=ORIENTED_EDGE ( 'NONE', *, *, #28157, .T. ) ;
#85721=CONICAL_SURFACE ( 'NONE', #102461, 0.09999999999999982514, 0.003490658503988666988 ) ;
#85722=EDGE_CURVE ( 'NONE', #29766, #113276, #8181, .T. ) ;
#85723=CIRCLE ( 'NONE', #125442, 0.09999999999999999167 ) ;
#85724=VERTEX_POINT ( 'NONE', #103275 ) ;
#85725=VERTEX_POINT ( 'NONE', #13580 ) ;
#85726=ADVANCED_FACE ( 'NONE', ( #113741 ), #24066, .T. ) ;
#85727=ORIENTED_EDGE ( 'NONE', *, *, #50090, .T. ) ;
#85728=EDGE_CURVE ( 'NONE', #105930, #14509, #123223, .T. ) ;
#85729=DIRECTION ( 'NONE',  ( -4.274815082592931898E-19, -0.9999939076577903929, -0.003490651415223739937 ) ) ;
#85730=DIRECTION ( 'NONE',  ( 0.000000000000000000, 1.000000000000000000, 0.000000000000000000 ) ) ;
#85731=AXIS2_PLACEMENT_3D ( 'NONE', #72581, #81113, #11712 ) ;
#85732=CARTESIAN_POINT ( 'NONE',  ( 1.049999999999952971, 2.500000000000000000, 6.148780366869520897 ) ) ;
#85733=FACE_OUTER_BOUND ( 'NONE', #96339, .T. ) ;
#85734=ADVANCED_FACE ( 'NONE', ( #18744 ), #112759, .T. ) ;
#85735=FACE_OUTER_BOUND ( 'NONE', #92286, .T. ) ;
#85736=EDGE_CURVE ( 'NONE', #33390, #102762, #46270, .T. ) ;
#85737=EDGE_LOOP ( 'NONE', ( #99076, #75301, #91960, #97803 ) ) ;
#85738=ADVANCED_FACE ( 'NONE', ( #96021 ), #56298, .T. ) ;
#85739=DIRECTION ( 'NONE',  ( 0.000000000000000000, -0.000000000000000000, 1.000000000000000000 ) ) ;
#85740=CONICAL_SURFACE ( 'NONE', #81552, 0.09999999999999999167, 0.003490658503988666988 ) ;
#85741=CARTESIAN_POINT ( 'NONE',  ( 13.09999999999990195, 2.500000000000000000, 4.776537180435972196 ) ) ;
#85744=CONICAL_SURFACE ( 'NONE', #62786, 0.1000000000000000472, 0.003490658503988666988 ) ;
#85745=ORIENTED_EDGE ( 'NONE', *, *, #91458, .T. ) ;
#85746=ORIENTED_EDGE ( 'NONE', *, *, #1535, .F. ) ;
#85747=DIRECTION ( 'NONE',  ( -0.000000000000000000, 1.000000000000000000, -0.000000000000000000 ) ) ;
#85748=CIRCLE ( 'NONE', #117129, 0.06509327318403745899 ) ;
#85749=CARTESIAN_POINT ( 'NONE',  ( -11.89999999999999680, 2.500000000000000000, -3.883716857408423984 ) ) ;
#85750=CARTESIAN_POINT ( 'NONE',  ( -3.150000000000029221, 12.50000000000000000, -1.818653347947326138 ) ) ;
#85751=AXIS2_PLACEMENT_3D ( 'NONE', #78579, #67412, #17689 ) ;
#85752=VERTEX_POINT ( 'NONE', #47577 ) ;
#85753=DIRECTION ( 'NONE',  ( 0.000000000000000000, 0.000000000000000000, 1.000000000000000000 ) ) ;
#85754=PLANE ( 'NONE',  #80955 ) ;
#85755=CARTESIAN_POINT ( 'NONE',  ( 13.29999999999989946, 2.500000000000000000, 0.09999999999999761857 ) ) ;
#85756=FACE_OUTER_BOUND ( 'NONE', #31902, .T. ) ;
#85757=FACE_OUTER_BOUND ( 'NONE', #83341, .T. ) ;
#85758=ORIENTED_EDGE ( 'NONE', *, *, #45918, .F. ) ;
#85759=DIRECTION ( 'NONE',  ( -1.000000000000000000, -0.000000000000000000, -0.000000000000000000 ) ) ;
#85760=EDGE_LOOP ( 'NONE', ( #87763, #52777 ) ) ;
#85761=EDGE_LOOP ( 'NONE', ( #44038, #99185, #61968, #93761 ) ) ;
#85762=VERTEX_POINT ( 'NONE', #27924 ) ;
#85763=CARTESIAN_POINT ( 'NONE',  ( -2.500000000000032419, 2.500000000000000000, -3.637306695894650055 ) ) ;
#85764=FACE_BOUND ( 'NONE', #52390, .T. ) ;
#85765=FACE_OUTER_BOUND ( 'NONE', #29166, .T. ) ;
#85766=DIRECTION ( 'NONE',  ( -4.274815082592931898E-19, -0.9999939076577903929, -0.003490651415223739937 ) ) ;
#85767=CARTESIAN_POINT ( 'NONE',  ( 4.599999999999940137, 12.50000000000000000, -5.022947341949754119 ) ) ;
#85768=VECTOR ( 'NONE', #23237, 1000.000000000000000 ) ;
#85769=EDGE_CURVE ( 'NONE', #39292, #78915, #14528, .T. ) ;
#85770=ORIENTED_EDGE ( 'NONE', *, *, #16692, .T. ) ;
#85771=EDGE_CURVE ( 'NONE', #33523, #3854, #35814, .T. ) ;
#85772=FACE_OUTER_BOUND ( 'NONE', #64070, .T. ) ;
#85773=AXIS2_PLACEMENT_3D ( 'NONE', #74441, #64608, #104537 ) ;
#85774=CARTESIAN_POINT ( 'NONE',  ( -3.350000000000028511, 2.500000000000000000, -2.957883832488653830 ) ) ;
#85775=CARTESIAN_POINT ( 'NONE',  ( -6.650000000000018119, 12.50000000000000000, -6.560283801567339701 ) ) ;
#85776=EDGE_CURVE ( 'NONE', #4707, #3076, #116289, .T. ) ;
#85777=DIRECTION ( 'NONE',  ( 0.000000000000000000, 0.000000000000000000, 1.000000000000000000 ) ) ;
#85779=CARTESIAN_POINT ( 'NONE',  ( 3.099999999999943245, 2.500000000000000000, 3.983716857408420076 ) ) ;
#85780=AXIS2_PLACEMENT_3D ( 'NONE', #52593, #24426, #74175 ) ;
#85781=VECTOR ( 'NONE', #60553, 1000.000000000000000 ) ;
#85782=CARTESIAN_POINT ( 'NONE',  ( 3.549999999999942091, 12.50000000000000000, 2.511473670974873507 ) ) ;
#85783=ADVANCED_FACE ( 'NONE', ( #65908 ), #77239, .T. ) ;
#85784=ORIENTED_EDGE ( 'NONE', *, *, #105746, .F. ) ;
#85785=DIRECTION ( 'NONE',  ( 0.000000000000000000, 1.000000000000000000, 0.000000000000000000 ) ) ;
#85786=EDGE_CURVE ( 'NONE', #67840, #58977, #16580, .T. ) ;
#85787=FACE_BOUND ( 'NONE', #103299, .T. ) ;
#85788=DIRECTION ( 'NONE',  ( -0.000000000000000000, -1.000000000000000000, -0.000000000000000000 ) ) ;
#85789=ADVANCED_FACE ( 'NONE', ( #67846 ), #115646, .T. ) ;
#85790=EDGE_CURVE ( 'NONE', #84307, #16039, #18650, .T. ) ;
#85791=ADVANCED_FACE ( 'NONE', ( #68487 ), #87602, .T. ) ;
#85792=ORIENTED_EDGE ( 'NONE', *, *, #105572, .F. ) ;
#85793=FACE_OUTER_BOUND ( 'NONE', #82942, .T. ) ;
#85794=DIRECTION ( 'NONE',  ( -0.000000000000000000, -1.000000000000000000, -0.000000000000000000 ) ) ;
#85795=ORIENTED_EDGE ( 'NONE', *, *, #122133, .T. ) ;
#85796=ORIENTED_EDGE ( 'NONE', *, *, #12480, .F. ) ;
#85798=EDGE_CURVE ( 'NONE', #27457, #99444, #77659, .T. ) ;
#85799=ORIENTED_EDGE ( 'NONE', *, *, #110620, .T. ) ;
#85801=DIRECTION ( 'NONE',  ( 0.000000000000000000, 0.000000000000000000, -1.000000000000000000 ) ) ;
#85802=DIRECTION ( 'NONE',  ( -0.000000000000000000, 1.000000000000000000, -0.000000000000000000 ) ) ;
#85803=CARTESIAN_POINT ( 'NONE',  ( 4.149999999999936406, 12.50000000000000000, 6.495190528383297135 ) ) ;
#85804=DIRECTION ( 'NONE',  ( 0.000000000000000000, 0.000000000000000000, -1.000000000000000000 ) ) ;
#85805=VECTOR ( 'NONE', #101519, 1000.000000000000000 ) ;
#85806=CONICAL_SURFACE ( 'NONE', #46115, 0.09999999999999982514, 0.003490658503988666988 ) ;
#85807=ORIENTED_EDGE ( 'NONE', *, *, #108774, .F. ) ;
#85808=EDGE_LOOP ( 'NONE', ( #50058, #104917 ) ) ;
#85809=LINE ( 'NONE', #17037, #15155 ) ;
#85810=DIRECTION ( 'NONE',  ( 0.000000000000000000, 0.000000000000000000, -1.000000000000000000 ) ) ;
#85811=CARTESIAN_POINT ( 'NONE',  ( 5.449999999999937117, 2.500000000000000000, -6.395190528383301931 ) ) ;
#85812=DIRECTION ( 'NONE',  ( 0.000000000000000000, 0.000000000000000000, -1.000000000000000000 ) ) ;
#85814=VERTEX_POINT ( 'NONE', #117560 ) ;
#85815=CARTESIAN_POINT ( 'NONE',  ( -11.25000000000000000, 2.500000000000000000, -2.757883832488650100 ) ) ;
#85816=VERTEX_POINT ( 'NONE', #8911 ) ;
#85817=DIRECTION ( 'NONE',  ( 0.000000000000000000, 1.000000000000000000, 0.000000000000000000 ) ) ;
#85818=DIRECTION ( 'NONE',  ( 0.000000000000000000, 0.000000000000000000, 1.000000000000000000 ) ) ;
#85819=AXIS2_PLACEMENT_3D ( 'NONE', #54065, #72426, #112346 ) ;
#85820=EDGE_LOOP ( 'NONE', ( #70274, #27026 ) ) ;
#85821=DIRECTION ( 'NONE',  ( 0.000000000000000000, -0.000000000000000000, 1.000000000000000000 ) ) ;
#85822=CARTESIAN_POINT ( 'NONE',  ( -4.150000000000025224, 2.500000000000000000, 5.802370205355744659 ) ) ;
#85823=CARTESIAN_POINT ( 'NONE',  ( 4.999999999999933387, 12.50000000000000000, 5.088040615133786027 ) ) ;
#85824=CARTESIAN_POINT ( 'NONE',  ( -3.350000000000028511, 12.50000000000000000, 2.857883832488649301 ) ) ;
#85825=CARTESIAN_POINT ( 'NONE',  ( -6.250000000000015987, 2.500000000000000000, 1.372243186433545370 ) ) ;
#85828=CARTESIAN_POINT ( 'NONE',  ( -5.200000000000020606, 2.500000000000000000, -0.4464101615137782142 ) ) ;
#85829=DIRECTION ( 'NONE',  ( -4.274815082592931898E-19, -0.9999939076577903929, -0.003490651415223739937 ) ) ;
#85830=AXIS2_PLACEMENT_3D ( 'NONE', #7833, #127619, #18937 ) ;
#85831=EDGE_LOOP ( 'NONE', ( #63689, #59998, #60527, #75479 ) ) ;
#85832=AXIS2_PLACEMENT_3D ( 'NONE', #80966, #120878, #31230 ) ;
#85833=ADVANCED_FACE ( 'NONE', ( #86172 ), #118238, .T. ) ;
#85834=VERTEX_POINT ( 'NONE', #7626 ) ;
#85835=CARTESIAN_POINT ( 'NONE',  ( -13.14999999999999147, 2.500000000000000000, 1.918653347947325338 ) ) ;
#85836=EDGE_LOOP ( 'NONE', ( #22101, #61458 ) ) ;
#85837=DIRECTION ( 'NONE',  ( 0.000000000000000000, -0.000000000000000000, 1.000000000000000000 ) ) ;
#85838=EDGE_LOOP ( 'NONE', ( #67310, #16194, #125926, #103772 ) ) ;
#85839=EDGE_LOOP ( 'NONE', ( #120679, #27893, #17148, #60564 ) ) ;
#85840=VERTEX_POINT ( 'NONE', #48873 ) ;
#85841=CARTESIAN_POINT ( 'NONE',  ( 13.09999999999990195, 2.500000000000000000, -3.983716857408426293 ) ) ;
#85842=VECTOR ( 'NONE', #29297, 1000.000000000000000 ) ;
#85843=CARTESIAN_POINT ( 'NONE',  ( -13.34999999999999076, 12.50000000000000000, 2.165063509461101265 ) ) ;
#85844=DIRECTION ( 'NONE',  ( -0.000000000000000000, -1.000000000000000000, -0.000000000000000000 ) ) ;
#85846=CARTESIAN_POINT ( 'NONE',  ( 12.09999999999990195, 2.500000000000000000, -0.7928203230275542301 ) ) ;
#85847=CARTESIAN_POINT ( 'NONE',  ( 5.849999999999931255, 12.50000000000000000, 2.857883832488649301 ) ) ;
#85848=EDGE_CURVE ( 'NONE', #100949, #75943, #119005, .T. ) ;
#85849=EDGE_LOOP ( 'NONE', ( #1608, #13269 ) ) ;
#85850=LINE ( 'NONE', #95696, #26794 ) ;
#85851=ORIENTED_EDGE ( 'NONE', *, *, #111840, .F. ) ;
#85853=ORIENTED_EDGE ( 'NONE', *, *, #83461, .F. ) ;
#85854=ORIENTED_EDGE ( 'NONE', *, *, #122559, .F. ) ;
#85855=DIRECTION ( 'NONE',  ( 0.000000000000000000, 0.000000000000000000, 1.000000000000000000 ) ) ;
#85856=VERTEX_POINT ( 'NONE', #16144 ) ;
#85857=VERTEX_POINT ( 'NONE', #56085 ) ;
#85858=CARTESIAN_POINT ( 'NONE',  ( 0.4499999999999552136, 2.500000000000000000, 6.495190528383297135 ) ) ;
#85859=DIRECTION ( 'NONE',  ( 0.000000000000000000, 0.000000000000000000, -1.000000000000000000 ) ) ;
#85860=DIRECTION ( 'NONE',  ( 0.000000000000000000, 0.000000000000000000, 1.000000000000000000 ) ) ;
#85861=DIRECTION ( 'NONE',  ( -0.000000000000000000, -1.000000000000000000, -0.000000000000000000 ) ) ;
#85862=DIRECTION ( 'NONE',  ( -4.274815082592931898E-19, -0.9999939076577903929, -0.003490651415223739937 ) ) ;
#85863=ORIENTED_EDGE ( 'NONE', *, *, #11586, .F. ) ;
#85864=AXIS2_PLACEMENT_3D ( 'NONE', #68980, #87953, #127907 ) ;
#85865=CARTESIAN_POINT ( 'NONE',  ( -4.800000000000024691, 12.50000000000000000, 0.3464101615137735735 ) ) ;
#85866=ORIENTED_EDGE ( 'NONE', *, *, #116127, .T. ) ;
#85867=PLANE ( 'NONE',  #44328 ) ;
#85868=EDGE_CURVE ( 'NONE', #110466, #38646, #6321, .T. ) ;
#85870=VERTEX_POINT ( 'NONE', #46941 ) ;
#85871=DIRECTION ( 'NONE',  ( 0.000000000000000000, 1.000000000000000000, 0.000000000000000000 ) ) ;
#85872=EDGE_LOOP ( 'NONE', ( #83398, #81383 ) ) ;
#85873=AXIS2_PLACEMENT_3D ( 'NONE', #39688, #37730, #88080 ) ;
#85874=ORIENTED_EDGE ( 'NONE', *, *, #124485, .T. ) ;
#85875=ADVANCED_FACE ( 'NONE', ( #31803 ), #35389, .T. ) ;
#85876=CARTESIAN_POINT ( 'NONE',  ( -8.300000000000011369, 12.50000000000000000, -4.330127018922201643 ) ) ;
#85877=DIRECTION ( 'NONE',  ( 0.000000000000000000, -0.000000000000000000, 1.000000000000000000 ) ) ;
#85878=CARTESIAN_POINT ( 'NONE',  ( -11.05000000000000249, 2.500000000000000000, -6.148780366869522673 ) ) ;
#85879=CARTESIAN_POINT ( 'NONE',  ( -10.20000000000000639, 12.50000000000000000, -3.918623584224384615 ) ) ;
#85880=EDGE_CURVE ( 'NONE', #82140, #122576, #6124, .T. ) ;
#85881=CARTESIAN_POINT ( 'NONE',  ( 11.24999999999990941, 2.500000000000000000, 7.088010851410848190 ) ) ;
#85882=ADVANCED_FACE ( 'NONE', ( #41642 ), #96023, .T. ) ;
#85883=EDGE_LOOP ( 'NONE', ( #119392, #55546 ) ) ;
#85884=DIRECTION ( 'NONE',  ( -0.000000000000000000, 1.000000000000000000, -0.000000000000000000 ) ) ;
#85885=CARTESIAN_POINT ( 'NONE',  ( 12.89999999999990266, 2.500000000000000000, 4.922947341949748257 ) ) ;
#85886=EDGE_CURVE ( 'NONE', #26403, #13366, #39617, .T. ) ;
#85887=DIRECTION ( 'NONE',  ( -0.000000000000000000, -1.000000000000000000, -0.000000000000000000 ) ) ;
#85888=EDGE_CURVE ( 'NONE', #106311, #113123, #81540, .T. ) ;
#85889=EDGE_CURVE ( 'NONE', #67958, #47787, #129306, .T. ) ;
#85890=FACE_OUTER_BOUND ( 'NONE', #75607, .T. ) ;
#85891=FACE_OUTER_BOUND ( 'NONE', #35552, .T. ) ;
#85892=ORIENTED_EDGE ( 'NONE', *, *, #44284, .T. ) ;
#85893=VECTOR ( 'NONE', #7757, 1000.000000000000000 ) ;
#85894=ORIENTED_EDGE ( 'NONE', *, *, #128504, .T. ) ;
#85895=CARTESIAN_POINT ( 'NONE',  ( -11.89999999999999503, 12.50000000000000000, 4.676537180435972552 ) ) ;
#85896=EDGE_CURVE ( 'NONE', #91980, #93976, #33149, .T. ) ;
#85897=VERTEX_POINT ( 'NONE', #90713 ) ;
#85898=DIRECTION ( 'NONE',  ( -0.000000000000000000, -1.000000000000000000, -0.000000000000000000 ) ) ;
#85899=VECTOR ( 'NONE', #10397, 1000.000000000000000 ) ;
#85900=CARTESIAN_POINT ( 'NONE',  ( 1.449999999999951328, 2.500000000000000000, -1.718653347947326049 ) ) ;
#85901=EDGE_CURVE ( 'NONE', #90888, #22290, #68920, .T. ) ;
#85904=CARTESIAN_POINT ( 'NONE',  ( 1.449999999999952216, 2.500000000000000000, -2.611473670974877592 ) ) ;
#85905=DIRECTION ( 'NONE',  ( 0.000000000000000000, -0.000000000000000000, 1.000000000000000000 ) ) ;
#85906=CARTESIAN_POINT ( 'NONE',  ( -8.550000000000009592, 2.500000000000000000, 6.841600689897072485 ) ) ;
#85907=EDGE_LOOP ( 'NONE', ( #36408, #5368, #60892, #24223 ) ) ;
#85908=AXIS2_PLACEMENT_3D ( 'NONE', #16354, #56296, #36686 ) ;
#85909=AXIS2_PLACEMENT_3D ( 'NONE', #91679, #81222, #43245 ) ;
#85910=DIRECTION ( 'NONE',  ( 0.000000000000000000, 0.000000000000000000, 1.000000000000000000 ) ) ;
#85911=FACE_OUTER_BOUND ( 'NONE', #11461, .T. ) ;
#85912=ORIENTED_EDGE ( 'NONE', *, *, #48385, .T. ) ;
#85913=LINE ( 'NONE', #40723, #56886 ) ;
#85914=FACE_OUTER_BOUND ( 'NONE', #112780, .T. ) ;
#85915=DIRECTION ( 'NONE',  ( 0.000000000000000000, 1.000000000000000000, 0.000000000000000000 ) ) ;
#85916=AXIS2_PLACEMENT_3D ( 'NONE', #120386, #50350, #128282 ) ;
#85917=ORIENTED_EDGE ( 'NONE', *, *, #110731, .T. ) ;
#85919=DIRECTION ( 'NONE',  ( 0.000000000000000000, 1.000000000000000000, 0.000000000000000000 ) ) ;
#85920=EDGE_LOOP ( 'NONE', ( #33685, #128640 ) ) ;
#85921=DIRECTION ( 'NONE',  ( 0.000000000000000000, 0.000000000000000000, 1.000000000000000000 ) ) ;
#85922=DIRECTION ( 'NONE',  ( -0.000000000000000000, 1.000000000000000000, -0.000000000000000000 ) ) ;
#85923=CIRCLE ( 'NONE', #48386, 0.1000000000000002554 ) ;
#85924=CARTESIAN_POINT ( 'NONE',  ( -14.59999999999998366, 2.500000000000000000, 0.09999999999999989453 ) ) ;
#85925=EDGE_CURVE ( 'NONE', #24108, #60798, #16667, .T. ) ;
#85926=VERTEX_POINT ( 'NONE', #377 ) ;
#85927=FACE_OUTER_BOUND ( 'NONE', #84590, .T. ) ;
#85928=ADVANCED_FACE ( 'NONE', ( #78976 ), #89847, .T. ) ;
#85929=CARTESIAN_POINT ( 'NONE',  ( -0.4000000000000331624, 2.500000000000000000, 0.000000000000000000 ) ) ;
#85930=AXIS2_PLACEMENT_3D ( 'NONE', #34547, #84254, #4383 ) ;
#85931=ORIENTED_EDGE ( 'NONE', *, *, #69863, .F. ) ;
#85932=EDGE_CURVE ( 'NONE', #120284, #99983, #81451, .T. ) ;
#85933=EDGE_LOOP ( 'NONE', ( #59974, #30279 ) ) ;
#85934=CARTESIAN_POINT ( 'NONE',  ( 1.649999999999949729, 2.500000000000000000, 7.288010851410849256 ) ) ;
#85935=ADVANCED_FACE ( 'NONE', ( #1041 ), #12484, .T. ) ;
#85936=EDGE_CURVE ( 'NONE', #45123, #5118, #109040, .T. ) ;
#85937=ORIENTED_EDGE ( 'NONE', *, *, #85936, .T. ) ;
#85938=DIRECTION ( 'NONE',  ( -0.000000000000000000, -1.000000000000000000, -0.000000000000000000 ) ) ;
#85939=CARTESIAN_POINT ( 'NONE',  ( -15.59999999999998010, 2.500000000000000000, 0.3464101615137759604 ) ) ;
#85940=VERTEX_POINT ( 'NONE', #61262 ) ;
#85941=DIRECTION ( 'NONE',  ( -0.000000000000000000, -1.000000000000000000, -0.000000000000000000 ) ) ;
#85942=DIRECTION ( 'NONE',  ( 0.000000000000000000, 0.000000000000000000, -1.000000000000000000 ) ) ;
#85943=EDGE_LOOP ( 'NONE', ( #62536, #1817 ) ) ;
#85944=ADVANCED_FACE ( 'NONE', ( #39064 ), #39713, .T. ) ;
#85945=DIRECTION ( 'NONE',  ( -0.000000000000000000, 1.000000000000000000, -0.000000000000000000 ) ) ;
#85946=DIRECTION ( 'NONE',  ( 0.000000000000000000, 0.000000000000000000, 1.000000000000000000 ) ) ;
#85947=CIRCLE ( 'NONE', #125659, 0.06509327318403745899 ) ;
#85948=DIRECTION ( 'NONE',  ( 0.000000000000000000, -0.000000000000000000, 1.000000000000000000 ) ) ;
#85949=DIRECTION ( 'NONE',  ( -0.000000000000000000, -1.000000000000000000, -0.000000000000000000 ) ) ;
#85950=AXIS2_PLACEMENT_3D ( 'NONE', #19206, #27116, #97144 ) ;
#85951=FACE_OUTER_BOUND ( 'NONE', #16792, .T. ) ;
#85952=CARTESIAN_POINT ( 'NONE',  ( -7.050000000000013145, 2.500000000000000000, 2.165063509461097713 ) ) ;
#85953=AXIS2_PLACEMENT_3D ( 'NONE', #104124, #102198, #74655 ) ;
#85954=ORIENTED_EDGE ( 'NONE', *, *, #120735, .F. ) ;
#85955=AXIS2_PLACEMENT_3D ( 'NONE', #125448, #126084, #35787 ) ;
#85956=EDGE_LOOP ( 'NONE', ( #89464, #90266 ) ) ;
#85957=EDGE_LOOP ( 'NONE', ( #89196, #107237 ) ) ;
#85958=EDGE_LOOP ( 'NONE', ( #65748, #107492, #59475, #40365 ) ) ;
#85959=DIRECTION ( 'NONE',  ( 0.000000000000000000, 0.000000000000000000, 1.000000000000000000 ) ) ;
#85960=CARTESIAN_POINT ( 'NONE',  ( -0.2000000000000339284, 12.50000000000000000, -0.4115034346978133639 ) ) ;
#85962=CARTESIAN_POINT ( 'NONE',  ( -8.350000000000008527, 2.500000000000000000, 5.802370205355744659 ) ) ;
#85964=FACE_BOUND ( 'NONE', #91314, .T. ) ;
#85965=ADVANCED_FACE ( 'NONE', ( #29861 ), #51452, .T. ) ;
#85966=CARTESIAN_POINT ( 'NONE',  ( -5.850000000000022737, 2.500000000000000000, -6.395190528383301931 ) ) ;
#85967=FACE_OUTER_BOUND ( 'NONE', #112999, .T. ) ;
#85968=CARTESIAN_POINT ( 'NONE',  ( -2.050000000000032685, 12.50000000000000000, -2.165063509461101710 ) ) ;
#85969=DIRECTION ( 'NONE',  ( -0.000000000000000000, -1.000000000000000000, -0.000000000000000000 ) ) ;
#85970=CARTESIAN_POINT ( 'NONE',  ( 16.87640210516338968, -2.500000000000000000, 4.436424697255031191 ) ) ;
#85971=CARTESIAN_POINT ( 'NONE',  ( -0.6000000000000383915, 2.500000000000000000, -4.576537180435977348 ) ) ;
#85972=CARTESIAN_POINT ( 'NONE',  ( -4.550000000000022915, 2.500000000000000000, 6.495190528383297135 ) ) ;
#85973=DIRECTION ( 'NONE',  ( 0.000000000000000000, 0.000000000000000000, 1.000000000000000000 ) ) ;
#85974=DIRECTION ( 'NONE',  ( -4.274815082592931898E-19, -0.9999939076577903929, -0.003490651415223739937 ) ) ;
#85975=CARTESIAN_POINT ( 'NONE',  ( 1.249999999999988454, 12.50000000000000000, -2.099970236277064473 ) ) ;
#85976=ORIENTED_EDGE ( 'NONE', *, *, #98746, .F. ) ;
#85977=ORIENTED_EDGE ( 'NONE', *, *, #41313, .F. ) ;
#85978=EDGE_CURVE ( 'NONE', #82935, #28339, #39716, .T. ) ;
#85979=VERTEX_POINT ( 'NONE', #99897 ) ;
#85980=ORIENTED_EDGE ( 'NONE', *, *, #63725, .T. ) ;
#85981=DIRECTION ( 'NONE',  ( -4.274815082592931898E-19, -0.9999939076577903929, -0.003490651415223739937 ) ) ;
#85982=ORIENTED_EDGE ( 'NONE', *, *, #44210, .F. ) ;
#85983=DIRECTION ( 'NONE',  ( 0.000000000000000000, -0.000000000000000000, 1.000000000000000000 ) ) ;
#85984=ORIENTED_EDGE ( 'NONE', *, *, #5457, .T. ) ;
#85985=EDGE_LOOP ( 'NONE', ( #113233, #94433, #41416, #6112 ) ) ;
#85986=DIRECTION ( 'NONE',  ( 0.000000000000000000, 0.000000000000000000, 1.000000000000000000 ) ) ;
#85988=LINE ( 'NONE', #125922, #124933 ) ;
#85989=CARTESIAN_POINT ( 'NONE',  ( -3.950000000000025491, 12.50000000000000000, 6.083687093685483660 ) ) ;
#85990=CARTESIAN_POINT ( 'NONE',  ( 8.099999999999923261, 12.50000000000000000, 3.983716857408420076 ) ) ;
#85991=CARTESIAN_POINT ( 'NONE',  ( -7.700000000000016165, 12.50000000000000000, 0.4115034346978109769 ) ) ;
#85992=EDGE_CURVE ( 'NONE', #104335, #92609, #10223, .T. ) ;
#85993=EDGE_LOOP ( 'NONE', ( #55262, #85443, #1668, #121441 ) ) ;
#85994=CONICAL_SURFACE ( 'NONE', #102719, 0.1000000000000002554, 0.003490658503988666988 ) ;
#85995=CIRCLE ( 'NONE', #63039, 0.09999999999999999167 ) ;
#85996=ORIENTED_EDGE ( 'NONE', *, *, #21313, .T. ) ;
#85997=ORIENTED_EDGE ( 'NONE', *, *, #13973, .T. ) ;
#85998=ORIENTED_EDGE ( 'NONE', *, *, #92290, .T. ) ;
#85999=FACE_OUTER_BOUND ( 'NONE', #96582, .T. ) ;
#86000=ORIENTED_EDGE ( 'NONE', *, *, #106322, .T. ) ;
#86001=VERTEX_POINT ( 'NONE', #112930 ) ;
#86002=AXIS2_PLACEMENT_3D ( 'NONE', #114414, #76435, #37167 ) ;
#86003=DIRECTION ( 'NONE',  ( 0.000000000000000000, 1.000000000000000000, 0.000000000000000000 ) ) ;
#86005=AXIS2_PLACEMENT_3D ( 'NONE', #119420, #29768, #80159 ) ;
#86006=DIRECTION ( 'NONE',  ( 0.000000000000000000, 0.000000000000000000, 1.000000000000000000 ) ) ;
#86007=CARTESIAN_POINT ( 'NONE',  ( -11.44999999999999751, 2.500000000000000000, 1.918653347947321564 ) ) ;
#86008=DIRECTION ( 'NONE',  ( 0.000000000000000000, 0.000000000000000000, 1.000000000000000000 ) ) ;
#86009=VECTOR ( 'NONE', #97346, 1000.000000000000000 ) ;
#86010=DIRECTION ( 'NONE',  ( 0.000000000000000000, 1.000000000000000000, 0.000000000000000000 ) ) ;
#86011=CARTESIAN_POINT ( 'NONE',  ( -3.100000000000028511, 12.50000000000000000, -4.741630453620015118 ) ) ;
#86012=ORIENTED_EDGE ( 'NONE', *, *, #23827, .F. ) ;
#86013=CARTESIAN_POINT ( 'NONE',  ( -13.09999999999999076, 2.500000000000000000, 4.083716857408421497 ) ) ;
#86014=EDGE_LOOP ( 'NONE', ( #72046, #19488, #112074, #78740 ) ) ;
#86015=DIRECTION ( 'NONE',  ( -0.000000000000000000, -1.000000000000000000, -0.000000000000000000 ) ) ;
#86016=ADVANCED_FACE ( 'NONE', ( #13427 ), #12777, .T. ) ;
#86017=ORIENTED_EDGE ( 'NONE', *, *, #121970, .T. ) ;
#86018=DIRECTION ( 'NONE',  ( -4.274815082592931898E-19, -0.9999939076577903929, -0.003490651415223739937 ) ) ;
#86019=CONICAL_SURFACE ( 'NONE', #73510, 0.1000000000000002554, 0.003490658503988666988 ) ;
#86020=CIRCLE ( 'NONE', #44263, 0.09999999999999982514 ) ;
#86021=FACE_OUTER_BOUND ( 'NONE', #109155, .T. ) ;
#86022=ORIENTED_EDGE ( 'NONE', *, *, #105688, .F. ) ;
#86023=CARTESIAN_POINT ( 'NONE',  ( -5.650000000000023448, 12.50000000000000000, -6.776507416713040577 ) ) ;
#86024=CARTESIAN_POINT ( 'NONE',  ( -11.44999999999999751, 2.500000000000000000, -2.511473670974873951 ) ) ;
#86025=VERTEX_POINT ( 'NONE', #84104 ) ;
#86026=EDGE_CURVE ( 'NONE', #91737, #8978, #44847, .T. ) ;
#86027=DIRECTION ( 'NONE',  ( -0.000000000000000000, 1.000000000000000000, -0.000000000000000000 ) ) ;
#86028=ORIENTED_EDGE ( 'NONE', *, *, #32919, .F. ) ;
#86029=EDGE_CURVE ( 'NONE', #45024, #8842, #39426, .T. ) ;
#86030=ADVANCED_FACE ( 'NONE', ( #93941 ), #34394, .T. ) ;
#86031=ORIENTED_EDGE ( 'NONE', *, *, #10650, .F. ) ;
#86032=PLANE ( 'NONE',  #79254 ) ;
#86033=DIRECTION ( 'NONE',  ( -0.000000000000000000, -1.000000000000000000, -0.000000000000000000 ) ) ;
#86034=EDGE_CURVE ( 'NONE', #96832, #104331, #124034, .T. ) ;
#86036=ADVANCED_FACE ( 'NONE', ( #74304 ), #95836, .T. ) ;
#86037=CARTESIAN_POINT ( 'NONE',  ( -6.249999999999984901, 12.50000000000000000, -6.430097255199264339 ) ) ;
#86038=FACE_OUTER_BOUND ( 'NONE', #19167, .T. ) ;
#86039=EDGE_CURVE ( 'NONE', #98143, #52604, #15350, .T. ) ;
#86040=DIRECTION ( 'NONE',  ( 0.000000000000000000, 0.000000000000000000, 1.000000000000000000 ) ) ;
#86042=AXIS2_PLACEMENT_3D ( 'NONE', #43161, #102685, #25404 ) ;
#86043=AXIS2_PLACEMENT_3D ( 'NONE', #97632, #58372, #36797 ) ;
#86044=ADVANCED_FACE ( 'NONE', ( #2310 ), #75187, .T. ) ;
#86045=EDGE_CURVE ( 'NONE', #69532, #87361, #22688, .T. ) ;
#86046=ORIENTED_EDGE ( 'NONE', *, *, #103334, .T. ) ;
#86047=EDGE_CURVE ( 'NONE', #100718, #15933, #62680, .T. ) ;
#86048=CARTESIAN_POINT ( 'NONE',  ( 2.049999999999950084, 2.500000000000000000, -2.165063509461101710 ) ) ;
#86049=AXIS2_PLACEMENT_3D ( 'NONE', #21542, #112509, #3832 ) ;
#86050=ADVANCED_FACE ( 'NONE', ( #82185 ), #122752, .T. ) ;
#86052=ORIENTED_EDGE ( 'NONE', *, *, #37293, .T. ) ;
#86053=VECTOR ( 'NONE', #104285, 1000.000000000000000 ) ;
#86054=DIRECTION ( 'NONE',  ( -0.000000000000000000, 1.000000000000000000, -0.000000000000000000 ) ) ;
#86055=CARTESIAN_POINT ( 'NONE',  ( 0.8499999999999553468, 2.500000000000000000, 1.472243186433545459 ) ) ;
#86056=DIRECTION ( 'NONE',  ( 0.000000000000000000, -0.9999939076577903929, 0.003490651415223739937 ) ) ;
#86057=EDGE_CURVE ( 'NONE', #16616, #65580, #33439, .T. ) ;
#86058=VERTEX_POINT ( 'NONE', #73008 ) ;
#86059=DIRECTION ( 'NONE',  ( -0.000000000000000000, -1.000000000000000000, -0.000000000000000000 ) ) ;
#86060=DIRECTION ( 'NONE',  ( -0.000000000000000000, 1.000000000000000000, -0.000000000000000000 ) ) ;
#86061=ORIENTED_EDGE ( 'NONE', *, *, #78889, .T. ) ;
#86062=DIRECTION ( 'NONE',  ( 0.000000000000000000, 0.000000000000000000, 1.000000000000000000 ) ) ;
#86063=ORIENTED_EDGE ( 'NONE', *, *, #12305, .T. ) ;
#86064=VERTEX_POINT ( 'NONE', #25184 ) ;
#86065=PLANE ( 'NONE',  #113716 ) ;
#86066=VERTEX_POINT ( 'NONE', #22636 ) ;
#86067=CARTESIAN_POINT ( 'NONE',  ( -5.200000000000025935, 2.500000000000000000, -3.883716857408426648 ) ) ;
#86068=LINE ( 'NONE', #14116, #42218 ) ;
#86069=LINE ( 'NONE', #126672, #35460 ) ;
#86070=AXIS2_PLACEMENT_3D ( 'NONE', #23279, #14097, #104423 ) ;
#86072=CIRCLE ( 'NONE', #98597, 0.09999999999999982514 ) ;
#86073=FACE_BOUND ( 'NONE', #10185, .T. ) ;
#86074=CARTESIAN_POINT ( 'NONE',  ( 13.34999999999990017, 2.500000000000000000, 1.472243186433545459 ) ) ;
#86075=EDGE_LOOP ( 'NONE', ( #77445, #23410, #115348, #51935 ) ) ;
#86076=DIRECTION ( 'NONE',  ( -0.000000000000000000, 1.000000000000000000, -0.000000000000000000 ) ) ;
#86077=CARTESIAN_POINT ( 'NONE',  ( -10.45000000000000462, 2.500000000000000000, -6.495190528383298911 ) ) ;
#86078=VERTEX_POINT ( 'NONE', #112295 ) ;
#86079=VECTOR ( 'NONE', #29063, 1000.000000000000000 ) ;
#86080=EDGE_CURVE ( 'NONE', #22999, #356, #102091, .T. ) ;
#86081=AXIS2_PLACEMENT_3D ( 'NONE', #101680, #83949, #36164 ) ;
#86082=AXIS2_PLACEMENT_3D ( 'NONE', #13451, #74322, #14726 ) ;
#86083=ORIENTED_EDGE ( 'NONE', *, *, #122241, .F. ) ;
#86084=EDGE_CURVE ( 'NONE', #97627, #5867, #103107, .T. ) ;
#86085=EDGE_LOOP ( 'NONE', ( #65546, #99856 ) ) ;
#86086=CARTESIAN_POINT ( 'NONE',  ( -0.6000000000000323963, 2.500000000000000000, -0.3464101615137759604 ) ) ;
#86087=DIRECTION ( 'NONE',  ( -0.000000000000000000, -1.000000000000000000, -0.000000000000000000 ) ) ;
#86089=DIRECTION ( 'NONE',  ( 0.000000000000000000, 0.000000000000000000, 1.000000000000000000 ) ) ;
#86090=FACE_BOUND ( 'NONE', #38502, .T. ) ;
#86091=ORIENTED_EDGE ( 'NONE', *, *, #88900, .T. ) ;
#86093=LINE ( 'NONE', #25917, #74067 ) ;
#86094=DIRECTION ( 'NONE',  ( 0.000000000000000000, 1.000000000000000000, 0.000000000000000000 ) ) ;
#86096=EDGE_CURVE ( 'NONE', #106091, #67575, #106568, .T. ) ;
#86097=CIRCLE ( 'NONE', #29691, 0.06509327318403745899 ) ;
#86098=CIRCLE ( 'NONE', #58942, 0.1000000000000002554 ) ;
#86099=AXIS2_PLACEMENT_3D ( 'NONE', #6918, #127378, #18046 ) ;
#86100=DIRECTION ( 'NONE',  ( -4.274815082592931898E-19, -0.9999939076577903929, -0.003490651415223739937 ) ) ;
#86101=DIRECTION ( 'NONE',  ( 0.000000000000000000, 1.000000000000000000, 0.000000000000000000 ) ) ;
#86102=DIRECTION ( 'NONE',  ( 0.000000000000000000, 0.000000000000000000, 1.000000000000000000 ) ) ;
#86103=VECTOR ( 'NONE', #107372, 1000.000000000000000 ) ;
#86104=CARTESIAN_POINT ( 'NONE',  ( -6.249999999999984901, 2.500000000000000000, -2.165063509461101710 ) ) ;
#86105=DIRECTION ( 'NONE',  ( 0.000000000000000000, 0.000000000000000000, 1.000000000000000000 ) ) ;
#86106=ORIENTED_EDGE ( 'NONE', *, *, #124437, .T. ) ;
#86107=AXIS2_PLACEMENT_3D ( 'NONE', #18992, #127045, #48473 ) ;
#86108=ORIENTED_EDGE ( 'NONE', *, *, #67709, .F. ) ;
#86109=ORIENTED_EDGE ( 'NONE', *, *, #109830, .T. ) ;
#86110=ORIENTED_EDGE ( 'NONE', *, *, #32658, .T. ) ;
#86112=DIRECTION ( 'NONE',  ( -4.274815082592931898E-19, -0.9999939076577903929, -0.003490651415223739937 ) ) ;
#86113=CARTESIAN_POINT ( 'NONE',  ( 9.999999999999952038, 2.500000000000000000, -2.276824562219559311E-15 ) ) ;
#86114=ORIENTED_EDGE ( 'NONE', *, *, #19094, .F. ) ;
#86115=FACE_BOUND ( 'NONE', #41479, .T. ) ;
#86116=DIRECTION ( 'NONE',  ( 0.000000000000000000, -0.9999939076577903929, 0.003490651415223739937 ) ) ;
#86117=DIRECTION ( 'NONE',  ( 0.000000000000000000, 1.000000000000000000, 0.000000000000000000 ) ) ;
#86118=FACE_OUTER_BOUND ( 'NONE', #66045, .T. ) ;
#86119=DIRECTION ( 'NONE',  ( 0.000000000000000000, -0.000000000000000000, 1.000000000000000000 ) ) ;
#86121=VERTEX_POINT ( 'NONE', #113578 ) ;
#86122=DIRECTION ( 'NONE',  ( 0.000000000000000000, 0.000000000000000000, -1.000000000000000000 ) ) ;
#86123=ORIENTED_EDGE ( 'NONE', *, *, #6971, .F. ) ;
#86124=ORIENTED_EDGE ( 'NONE', *, *, #54550, .F. ) ;
#86125=AXIS2_PLACEMENT_3D ( 'NONE', #81607, #24632, #101901 ) ;
#86126=VERTEX_POINT ( 'NONE', #8124 ) ;
#86127=CIRCLE ( 'NONE', #111261, 0.1000000000000002554 ) ;
#86128=DIRECTION ( 'NONE',  ( 0.000000000000000000, 1.000000000000000000, 0.000000000000000000 ) ) ;
#86129=CONICAL_SURFACE ( 'NONE', #104912, 0.09999999999999999167, 0.003490658503988666988 ) ;
#86130=CARTESIAN_POINT ( 'NONE',  ( -7.500000000000016875, 12.50000000000000000, 0.6928203230275494784 ) ) ;
#86131=FACE_OUTER_BOUND ( 'NONE', #11261, .T. ) ;
#86132=ORIENTED_EDGE ( 'NONE', *, *, #6989, .F. ) ;
#86133=CARTESIAN_POINT ( 'NONE',  ( 15.62920359459757336, 2.499999999999999556, -5.623946225393742004 ) ) ;
#86134=CARTESIAN_POINT ( 'NONE',  ( -5.850000000000018296, 12.50000000000000000, 7.188010851410848723 ) ) ;
#86135=AXIS2_PLACEMENT_3D ( 'NONE', #75785, #17501, #104604 ) ;
#86136=VECTOR ( 'NONE', #95569, 1000.000000000000000 ) ;
#86137=CIRCLE ( 'NONE', #35999, 0.09999999999999999167 ) ;
#86138=CARTESIAN_POINT ( 'NONE',  ( -4.200000000000029488, 2.500000000000000000, -4.430127018922202176 ) ) ;
#86140=CARTESIAN_POINT ( 'NONE',  ( 11.04999999999991012, 12.50000000000000000, -1.883746621131363597 ) ) ;
#86141=CONICAL_SURFACE ( 'NONE', #464, 0.1000000000000000472, 0.003490658503988666988 ) ;
#86142=EDGE_CURVE ( 'NONE', #41595, #55841, #56571, .T. ) ;
#86143=CONICAL_SURFACE ( 'NONE', #100823, 0.09999999999999999167, 0.003490658503988666988 ) ;
#86144=CARTESIAN_POINT ( 'NONE',  ( -11.89999999999999503, 2.500000000000000000, 4.576537180435972019 ) ) ;
#86145=EDGE_CURVE ( 'NONE', #46062, #122449, #112564, .T. ) ;
#86147=CARTESIAN_POINT ( 'NONE',  ( -5.850000000000018296, 2.500000000000000000, 7.188010851410848723 ) ) ;
#86148=AXIS2_PLACEMENT_3D ( 'NONE', #102622, #12943, #60782 ) ;
#86149=ORIENTED_EDGE ( 'NONE', *, *, #73607, .F. ) ;
#86150=ORIENTED_EDGE ( 'NONE', *, *, #48870, .T. ) ;
#86152=DIRECTION ( 'NONE',  ( 0.000000000000000000, -0.000000000000000000, 1.000000000000000000 ) ) ;
#86153=DIRECTION ( 'NONE',  ( 0.000000000000000000, 0.000000000000000000, 1.000000000000000000 ) ) ;
#86154=EDGE_CURVE ( 'NONE', #79643, #27571, #6811, .T. ) ;
#86155=ORIENTED_EDGE ( 'NONE', *, *, #15547, .F. ) ;
#86156=VERTEX_POINT ( 'NONE', #68339 ) ;
#86157=DIRECTION ( 'NONE',  ( 0.000000000000000000, 0.000000000000000000, 1.000000000000000000 ) ) ;
#86158=CARTESIAN_POINT ( 'NONE',  ( 43.29532267389756583, 3.510960536759776485, -3.940524368371014052 ) ) ;
#86159=FACE_OUTER_BOUND ( 'NONE', #32756, .T. ) ;
#86160=ORIENTED_EDGE ( 'NONE', *, *, #3647, .F. ) ;
#86161=ORIENTED_EDGE ( 'NONE', *, *, #92500, .F. ) ;
#86162=DIRECTION ( 'NONE',  ( 0.000000000000000000, 0.000000000000000000, 1.000000000000000000 ) ) ;
#86163=AXIS2_PLACEMENT_3D ( 'NONE', #916, #79492, #108289 ) ;
#86164=EDGE_LOOP ( 'NONE', ( #118341, #85708, #2547, #54781 ) ) ;
#86165=LINE ( 'NONE', #67161, #58292 ) ;
#86166=CARTESIAN_POINT ( 'NONE',  ( -11.84999999999999609, 12.50000000000000000, 6.906693963081109722 ) ) ;
#86167=ORIENTED_EDGE ( 'NONE', *, *, #8514, .T. ) ;
#86168=DIRECTION ( 'NONE',  ( -0.000000000000000000, 1.000000000000000000, -0.000000000000000000 ) ) ;
#86169=ADVANCED_FACE ( 'NONE', ( #108263 ), #56107, .T. ) ;
#86170=DIRECTION ( 'NONE',  ( 0.000000000000000000, 0.000000000000000000, 1.000000000000000000 ) ) ;
#86171=DIRECTION ( 'NONE',  ( -0.000000000000000000, -1.000000000000000000, -0.000000000000000000 ) ) ;
#86172=FACE_OUTER_BOUND ( 'NONE', #66468, .T. ) ;
#86173=CONICAL_SURFACE ( 'NONE', #69461, 0.1000000000000000472, 0.003490658503988666988 ) ;
#86174=VERTEX_POINT ( 'NONE', #95874 ) ;
#86175=VECTOR ( 'NONE', #118060, 1000.000000000000000 ) ;
#86176=AXIS2_PLACEMENT_3D ( 'NONE', #30220, #10540, #30861 ) ;
#86177=EDGE_CURVE ( 'NONE', #49853, #92039, #116785, .T. ) ;
#86178=CARTESIAN_POINT ( 'NONE',  ( 7.099999999999927702, 2.500000000000000000, 5.022947341949748790 ) ) ;
#86179=FACE_OUTER_BOUND ( 'NONE', #4377, .T. ) ;
#86180=EDGE_LOOP ( 'NONE', ( #3797, #122709, #29793, #89476 ) ) ;
#86181=ORIENTED_EDGE ( 'NONE', *, *, #94951, .F. ) ;
#86182=EDGE_CURVE ( 'NONE', #103260, #59034, #127277, .T. ) ;
#86183=EDGE_CURVE ( 'NONE', #65479, #93927, #121154, .T. ) ;
#86185=FACE_OUTER_BOUND ( 'NONE', #105673, .T. ) ;
#86186=DIRECTION ( 'NONE',  ( -0.000000000000000000, 1.000000000000000000, -0.000000000000000000 ) ) ;
#86188=FACE_OUTER_BOUND ( 'NONE', #27950, .T. ) ;
#86189=EDGE_CURVE ( 'NONE', #45669, #73196, #76239, .T. ) ;
#86190=CARTESIAN_POINT ( 'NONE',  ( -5.000000000000022204, 12.50000000000000000, -0.6928203230275541413 ) ) ;
#86191=LINE ( 'NONE', #46954, #92429 ) ;
#86192=VECTOR ( 'NONE', #85154, 1000.000000000000000 ) ;
#86193=CARTESIAN_POINT ( 'NONE',  ( 16.98713586915519969, 1.503435535904362075, -5.629434499184647223 ) ) ;
#86194=AXIS2_PLACEMENT_3D ( 'NONE', #47728, #69272, #68641 ) ;
#86195=CARTESIAN_POINT ( 'NONE',  ( 9.399999999999915090, 12.50000000000000000, -3.983716857408426293 ) ) ;
#86196=AXIS2_PLACEMENT_3D ( 'NONE', #120489, #61585, #101499 ) ;
#86197=CONICAL_SURFACE ( 'NONE', #46493, 0.09999999999999999167, 0.003490658503988666988 ) ;
#86198=CARTESIAN_POINT ( 'NONE',  ( 9.799999999999915445, 12.50000000000000000, -4.676537180435977881 ) ) ;
#86199=EDGE_CURVE ( 'NONE', #3943, #13317, #125358, .T. ) ;
#86200=EDGE_CURVE ( 'NONE', #35689, #87216, #16642, .T. ) ;
#86201=AXIS2_PLACEMENT_3D ( 'NONE', #52323, #43810, #42524 ) ;
#86202=PLANE ( 'NONE',  #29226 ) ;
#86203=ORIENTED_EDGE ( 'NONE', *, *, #5208, .F. ) ;
#86204=EDGE_CURVE ( 'NONE', #29164, #20699, #16482, .T. ) ;
#86205=AXIS2_PLACEMENT_3D ( 'NONE', #100773, #102087, #13032 ) ;
#86206=ORIENTED_EDGE ( 'NONE', *, *, #40080, .T. ) ;
#86207=CARTESIAN_POINT ( 'NONE',  ( 14.59999999999989484, 12.50000000000000000, -0.06509327318403970719 ) ) ;
#86208=ORIENTED_EDGE ( 'NONE', *, *, #44201, .F. ) ;
#86209=EDGE_CURVE ( 'NONE', #53658, #11186, #60346, .T. ) ;
#86210=CARTESIAN_POINT ( 'NONE',  ( -11.84999999999999609, 2.500000000000000000, 1.818653347947321475 ) ) ;
#86211=CARTESIAN_POINT ( 'NONE',  ( -0.8500000000000390576, 2.500000000000000000, -6.495190528383302464 ) ) ;
#86212=DIRECTION ( 'NONE',  ( 0.000000000000000000, 1.000000000000000000, 0.000000000000000000 ) ) ;
#86213=ADVANCED_FACE ( 'NONE', ( #126631 ), #115486, .T. ) ;
#86214=VERTEX_POINT ( 'NONE', #118080 ) ;
#86215=LINE ( 'NONE', #26033, #105113 ) ;
#86217=DIRECTION ( 'NONE',  ( -0.000000000000000000, -1.000000000000000000, -0.000000000000000000 ) ) ;
#86218=ORIENTED_EDGE ( 'NONE', *, *, #113412, .T. ) ;
#86219=AXIS2_PLACEMENT_3D ( 'NONE', #40032, #2017, #72707 ) ;
#86220=DIRECTION ( 'NONE',  ( 0.000000000000000000, 0.000000000000000000, 1.000000000000000000 ) ) ;
#86221=ORIENTED_EDGE ( 'NONE', *, *, #87247, .T. ) ;
#86222=ORIENTED_EDGE ( 'NONE', *, *, #121200, .T. ) ;
#86223=ORIENTED_EDGE ( 'NONE', *, *, #97607, .F. ) ;
#86224=AXIS2_PLACEMENT_3D ( 'NONE', #107703, #86759, #8197 ) ;
#86225=ORIENTED_EDGE ( 'NONE', *, *, #13929, .F. ) ;
#86226=DIRECTION ( 'NONE',  ( 0.000000000000000000, 1.000000000000000000, 0.000000000000000000 ) ) ;
#86227=CIRCLE ( 'NONE', #65300, 0.06509327318403745899 ) ;
#86228=DIRECTION ( 'NONE',  ( 0.000000000000000000, -0.9999939076577903929, 0.003490651415223739937 ) ) ;
#86229=DIRECTION ( 'NONE',  ( 0.000000000000000000, 0.000000000000000000, 1.000000000000000000 ) ) ;
#86230=CARTESIAN_POINT ( 'NONE',  ( -4.150000000000025224, 12.50000000000000000, 6.560283801567334372 ) ) ;
#86231=CIRCLE ( 'NONE', #77835, 0.1000000000000002554 ) ;
#86232=ORIENTED_EDGE ( 'NONE', *, *, #95683, .T. ) ;
#86233=VECTOR ( 'NONE', #8452, 1000.000000000000000 ) ;
#86234=CONICAL_SURFACE ( 'NONE', #107170, 0.1000000000000002554, 0.003490658503988666988 ) ;
#86235=LINE ( 'NONE', #126180, #46127 ) ;
#86236=AXIS2_PLACEMENT_3D ( 'NONE', #71514, #69583, #109518 ) ;
#86237=ORIENTED_EDGE ( 'NONE', *, *, #69188, .T. ) ;
#86238=CARTESIAN_POINT ( 'NONE',  ( 59.88087687688727812, -3.776023963367705516, -4.996435080130480877 ) ) ;
#86239=CARTESIAN_POINT ( 'NONE',  ( 15.23091471310473999, -2.500000000000513367, -7.179421168902700323 ) ) ;
#86240=CIRCLE ( 'NONE', #6710, 0.06509327318403745899 ) ;
#86241=CARTESIAN_POINT ( 'NONE',  ( 2.099999999999950351, 2.500000000000000000, -4.430127018922202176 ) ) ;
#86242=CARTESIAN_POINT ( 'NONE',  ( 18.27284318114671180, -0.4998542452747786746, 4.791717918553223932 ) ) ;
#86243=CIRCLE ( 'NONE', #57000, 0.06509327318403745899 ) ;
#86244=EDGE_LOOP ( 'NONE', ( #54199, #37808, #64665, #37045 ) ) ;
#86245=EDGE_CURVE ( 'NONE', #63643, #68589, #116748, .T. ) ;
#86246=ORIENTED_EDGE ( 'NONE', *, *, #2981, .T. ) ;
#86247=ADVANCED_FACE ( 'NONE', ( #95234 ), #66572, .T. ) ;
#86248=EDGE_LOOP ( 'NONE', ( #100946, #116907, #69725, #66451 ) ) ;
#86249=PLANE ( 'NONE',  #48193 ) ;
#86250=CARTESIAN_POINT ( 'NONE',  ( 9.549999999999915445, 12.50000000000000000, -2.165063509461101710 ) ) ;
#86251=CARTESIAN_POINT ( 'NONE',  ( -9.150000000000009237, 2.500000000000000000, -7.088010851410848190 ) ) ;
#86252=FACE_BOUND ( 'NONE', #89056, .T. ) ;
#86253=CARTESIAN_POINT ( 'NONE',  ( 5.849999999999933031, 12.50000000000000000, 7.188010851410848723 ) ) ;
#86254=CARTESIAN_POINT ( 'NONE',  ( -2.499999999999996003, 12.50000000000000000, -4.330127018922201643 ) ) ;
#86255=CARTESIAN_POINT ( 'NONE',  ( -4.293440603042597559E-14, 12.50000000000000000, 5.022947341949748790 ) ) ;
#86256=CARTESIAN_POINT ( 'NONE',  ( -7.500000000000011546, 2.500000000000000000, 3.637306695894644726 ) ) ;
#86257=AXIS2_PLACEMENT_3D ( 'NONE', #83376, #44084, #113465 ) ;
#86259=DIRECTION ( 'NONE',  ( -0.000000000000000000, -1.000000000000000000, -0.000000000000000000 ) ) ;
#86260=LINE ( 'NONE', #7705, #57415 ) ;
#86261=AXIS2_PLACEMENT_3D ( 'NONE', #126498, #95105, #85905 ) ;
#86262=CIRCLE ( 'NONE', #27780, 0.1000000000000002554 ) ;
#86263=AXIS2_PLACEMENT_3D ( 'NONE', #21758, #101608, #51863 ) ;
#86264=DIRECTION ( 'NONE',  ( 0.000000000000000000, 0.000000000000000000, 1.000000000000000000 ) ) ;
#86265=ORIENTED_EDGE ( 'NONE', *, *, #122429, .T. ) ;
#86266=ORIENTED_EDGE ( 'NONE', *, *, #75507, .T. ) ;
#86267=EDGE_LOOP ( 'NONE', ( #22917, #8426, #94340, #87521 ) ) ;
#86268=EDGE_LOOP ( 'NONE', ( #30769, #64474, #128690 ) ) ;
#86269=LINE ( 'NONE', #106564, #33995 ) ;
#86270=FACE_BOUND ( 'NONE', #113436, .T. ) ;
#86271=CONICAL_SURFACE ( 'NONE', #84221, 0.1000000000000002554, 0.003490658503988666988 ) ;
#86272=CARTESIAN_POINT ( 'NONE',  ( -11.84999999999999609, 2.500000000000000000, 6.148780366869520897 ) ) ;
#86274=LINE ( 'NONE', #88197, #43593 ) ;
#86275=CIRCLE ( 'NONE', #67489, 0.06509327318403745899 ) ;
#86276=AXIS2_PLACEMENT_3D ( 'NONE', #86554, #127143, #37479 ) ;
#86277=EDGE_LOOP ( 'NONE', ( #94628, #64376, #115474, #53063 ) ) ;
#86278=DIRECTION ( 'NONE',  ( 0.000000000000000000, -0.9999939076577903929, 0.003490651415223739937 ) ) ;
#86279=CARTESIAN_POINT ( 'NONE',  ( -8.950000000000008171, 12.50000000000000000, -2.576566944158915184 ) ) ;
#86280=ORIENTED_EDGE ( 'NONE', *, *, #58265, .F. ) ;
#86281=CIRCLE ( 'NONE', #31934, 0.06509327318403745899 ) ;
#86282=CARTESIAN_POINT ( 'NONE',  ( -10.85000000000000142, 12.50000000000000000, -2.857883832488649745 ) ) ;
#86283=CARTESIAN_POINT ( 'NONE',  ( -5.400000000000019895, 2.500000000000000000, -0.6928203230275541413 ) ) ;
#86284=CIRCLE ( 'NONE', #96750, 0.1000000000000000472 ) ;
#86285=EDGE_CURVE ( 'NONE', #126271, #81614, #33251, .T. ) ;
#86286=AXIS2_PLACEMENT_3D ( 'NONE', #120739, #29785, #39636 ) ;
#86287=AXIS2_PLACEMENT_3D ( 'NONE', #55609, #14378, #105359 ) ;
#86288=VECTOR ( 'NONE', #75853, 1000.000000000000000 ) ;
#86289=ORIENTED_EDGE ( 'NONE', *, *, #47209, .F. ) ;
#86290=FACE_OUTER_BOUND ( 'NONE', #72178, .T. ) ;
#86291=LINE ( 'NONE', #116399, #76775 ) ;
#86292=AXIS2_PLACEMENT_3D ( 'NONE', #1763, #12860, #121538 ) ;
#86294=ORIENTED_EDGE ( 'NONE', *, *, #37621, .T. ) ;
#86295=DIRECTION ( 'NONE',  ( -0.000000000000000000, 1.000000000000000000, -0.000000000000000000 ) ) ;
#86296=AXIS2_PLACEMENT_3D ( 'NONE', #26745, #107877, #87585 ) ;
#86297=DIRECTION ( 'NONE',  ( 0.000000000000000000, 0.000000000000000000, 1.000000000000000000 ) ) ;
#86298=ORIENTED_EDGE ( 'NONE', *, *, #12141, .F. ) ;
#86299=DIRECTION ( 'NONE',  ( -0.000000000000000000, 1.000000000000000000, -0.000000000000000000 ) ) ;
#86300=ORIENTED_EDGE ( 'NONE', *, *, #89578, .T. ) ;
#86301=ADVANCED_FACE ( 'NONE', ( #46125 ), #18558, .T. ) ;
#86302=EDGE_LOOP ( 'NONE', ( #36016, #9266, #45456, #1809 ) ) ;
#86303=EDGE_CURVE ( 'NONE', #58472, #21571, #110497, .T. ) ;
#86304=CARTESIAN_POINT ( 'NONE',  ( -9.800000000000006040, 2.500000000000000000, -4.676537180435974328 ) ) ;
#86305=VERTEX_POINT ( 'NONE', #58541 ) ;
#86306=CARTESIAN_POINT ( 'NONE',  ( 4.349999999999939249, 2.500000000000000000, 2.611473670974873151 ) ) ;
#86307=DIRECTION ( 'NONE',  ( 0.000000000000000000, 0.000000000000000000, 1.000000000000000000 ) ) ;
#86309=CARTESIAN_POINT ( 'NONE',  ( -1.650000000000034328, 2.500000000000000000, -7.188010851410854052 ) ) ;
#86310=CARTESIAN_POINT ( 'NONE',  ( -12.89999999999999325, 2.500000000000000000, 0.7928203230275536750 ) ) ;
#86311=DIRECTION ( 'NONE',  ( 0.000000000000000000, -0.000000000000000000, 1.000000000000000000 ) ) ;
#86312=DIRECTION ( 'NONE',  ( 0.000000000000000000, -0.9999939076577903929, 0.003490651415223739937 ) ) ;
#86313=AXIS2_PLACEMENT_3D ( 'NONE', #39256, #7169, #47764 ) ;
#86314=DIRECTION ( 'NONE',  ( 0.000000000000000000, 0.000000000000000000, -1.000000000000000000 ) ) ;
#86315=EDGE_CURVE ( 'NONE', #26633, #55841, #91718, .T. ) ;
#86316=CARTESIAN_POINT ( 'NONE',  ( -1.450000000000035927, 2.500000000000000000, -6.248780366869526759 ) ) ;
#86317=ORIENTED_EDGE ( 'NONE', *, *, #8475, .T. ) ;
#86318=ORIENTED_EDGE ( 'NONE', *, *, #13931, .F. ) ;
#86319=DIRECTION ( 'NONE',  ( 0.000000000000000000, -0.000000000000000000, 1.000000000000000000 ) ) ;
#86320=AXIS2_PLACEMENT_3D ( 'NONE', #102510, #101226, #81577 ) ;
#86321=AXIS2_PLACEMENT_3D ( 'NONE', #81155, #30132, #51696 ) ;
#86322=CARTESIAN_POINT ( 'NONE',  ( 20.37757664703727656, -0.6627606010238995538, 4.188167776336781500 ) ) ;
#86323=AXIS2_PLACEMENT_3D ( 'NONE', #67967, #47707, #127547 ) ;
#86324=CIRCLE ( 'NONE', #11105, 0.1000000000000002554 ) ;
#86325=DIRECTION ( 'NONE',  ( 0.000000000000000000, 1.000000000000000000, 0.000000000000000000 ) ) ;
#86326=EDGE_LOOP ( 'NONE', ( #123072, #66644, #32636, #108594 ) ) ;
#86327=EDGE_LOOP ( 'NONE', ( #62744, #23736 ) ) ;
#86328=ORIENTED_EDGE ( 'NONE', *, *, #37850, .T. ) ;
#86329=CARTESIAN_POINT ( 'NONE',  ( -11.04999999999999893, 12.50000000000000000, 6.148780366869520009 ) ) ;
#86330=DIRECTION ( 'NONE',  ( 0.000000000000000000, 0.000000000000000000, 1.000000000000000000 ) ) ;
#86331=AXIS2_PLACEMENT_3D ( 'NONE', #67538, #57755, #117939 ) ;
#86332=VECTOR ( 'NONE', #58076, 1000.000000000000000 ) ;
#86333=DIRECTION ( 'NONE',  ( 0.000000000000000000, -0.9999939076577903929, 0.003490651415223739937 ) ) ;
#86335=CARTESIAN_POINT ( 'NONE',  ( 3.149999999999944400, 2.500000000000000000, 1.818653347947321475 ) ) ;
#86337=AXIS2_PLACEMENT_3D ( 'NONE', #23378, #32599, #13558 ) ;
#86338=DIRECTION ( 'NONE',  ( 0.000000000000000000, 1.000000000000000000, 0.000000000000000000 ) ) ;
#86339=DIRECTION ( 'NONE',  ( 0.000000000000000000, 0.000000000000000000, 1.000000000000000000 ) ) ;
#86340=AXIS2_PLACEMENT_3D ( 'NONE', #90858, #23392, #62700 ) ;
#86341=DIRECTION ( 'NONE',  ( -0.000000000000000000, -1.000000000000000000, -0.000000000000000000 ) ) ;
#86342=AXIS2_PLACEMENT_3D ( 'NONE', #98284, #100235, #10541 ) ;
#86343=ORIENTED_EDGE ( 'NONE', *, *, #118017, .T. ) ;
#86344=EDGE_CURVE ( 'NONE', #67419, #107723, #56197, .T. ) ;
#86345=CARTESIAN_POINT ( 'NONE',  ( -4.800000000000022915, 12.50000000000000000, 4.048810130592458201 ) ) ;
#86346=EDGE_LOOP ( 'NONE', ( #51649, #13345 ) ) ;
#86347=ORIENTED_EDGE ( 'NONE', *, *, #43197, .T. ) ;
#86348=EDGE_CURVE ( 'NONE', #128842, #77757, #104242, .T. ) ;
#86350=CARTESIAN_POINT ( 'NONE',  ( 7.949999999999925571, 12.50000000000000000, 2.165063509461097713 ) ) ;
#86351=DIRECTION ( 'NONE',  ( 0.000000000000000000, 0.000000000000000000, 1.000000000000000000 ) ) ;
#86352=EDGE_CURVE ( 'NONE', #44450, #53076, #110835, .T. ) ;
#86353=CIRCLE ( 'NONE', #65429, 0.1000000000000002554 ) ;
#86354=DIRECTION ( 'NONE',  ( 0.000000000000000000, 0.000000000000000000, 1.000000000000000000 ) ) ;
#86355=DIRECTION ( 'NONE',  ( 0.000000000000000000, 0.000000000000000000, 1.000000000000000000 ) ) ;
#86356=CARTESIAN_POINT ( 'NONE',  ( 2.699999999999945555, 2.500000000000000000, 3.983716857408420076 ) ) ;
#86357=DIRECTION ( 'NONE',  ( 0.000000000000000000, -0.000000000000000000, 1.000000000000000000 ) ) ;
#86358=ORIENTED_EDGE ( 'NONE', *, *, #60380, .T. ) ;
#86359=DIRECTION ( 'NONE',  ( 0.000000000000000000, 0.000000000000000000, 1.000000000000000000 ) ) ;
#86360=EDGE_CURVE ( 'NONE', #35274, #40007, #61102, .T. ) ;
#86361=EDGE_CURVE ( 'NONE', #125999, #65236, #81260, .T. ) ;
#86362=EDGE_CURVE ( 'NONE', #30351, #25527, #11356, .T. ) ;
#86363=EDGE_CURVE ( 'NONE', #26544, #118638, #93782, .T. ) ;
#86364=AXIS2_PLACEMENT_3D ( 'NONE', #83677, #113127, #94780 ) ;
#86365=DIRECTION ( 'NONE',  ( 0.000000000000000000, 0.000000000000000000, -1.000000000000000000 ) ) ;
#86367=VERTEX_POINT ( 'NONE', #83168 ) ;
#86368=AXIS2_PLACEMENT_3D ( 'NONE', #74715, #123796, #56351 ) ;
#86369=VERTEX_POINT ( 'NONE', #98428 ) ;
#86370=EDGE_CURVE ( 'NONE', #122996, #98982, #8086, .T. ) ;
#86371=ORIENTED_EDGE ( 'NONE', *, *, #106482, .T. ) ;
#86372=ORIENTED_EDGE ( 'NONE', *, *, #18403, .F. ) ;
#86373=VECTOR ( 'NONE', #1909, 1000.000000000000000 ) ;
#86375=FACE_OUTER_BOUND ( 'NONE', #34666, .T. ) ;
#86376=CIRCLE ( 'NONE', #111515, 0.06509327318403745899 ) ;
#86377=ADVANCED_FACE ( 'NONE', ( #73323 ), #47816, .T. ) ;
#86378=AXIS2_PLACEMENT_3D ( 'NONE', #26605, #88069, #99221 ) ;
#86379=ORIENTED_EDGE ( 'NONE', *, *, #74426, .T. ) ;
#86380=CARTESIAN_POINT ( 'NONE',  ( 12.69999999999989981, 2.500000000000000000, -0.3464101615137783474 ) ) ;
#86381=CONICAL_SURFACE ( 'NONE', #29968, 0.09999999999999982514, 0.003490658503988666988 ) ;
#86382=CARTESIAN_POINT ( 'NONE',  ( 17.50000000000000000, 0.9166666666666685170, -2.864912725862979848 ) ) ;
#86383=DIRECTION ( 'NONE',  ( 0.000000000000000000, 1.000000000000000000, 0.000000000000000000 ) ) ;
#86384=ORIENTED_EDGE ( 'NONE', *, *, #16294, .T. ) ;
#86385=FACE_OUTER_BOUND ( 'NONE', #64204, .T. ) ;
#86386=DIRECTION ( 'NONE',  ( 0.000000000000000000, -0.9999939076577903929, 0.003490651415223739937 ) ) ;
#86387=EDGE_LOOP ( 'NONE', ( #117701, #94652, #24200, #38230 ) ) ;
#86388=CONICAL_SURFACE ( 'NONE', #63418, 0.1000000000000002554, 0.003490658503988666988 ) ;
#86389=CIRCLE ( 'NONE', #38293, 10.00000000000000000 ) ;
#86390=ORIENTED_EDGE ( 'NONE', *, *, #99675, .F. ) ;
#86391=EDGE_LOOP ( 'NONE', ( #106307, #25259, #59588, #88366 ) ) ;
#86392=FACE_OUTER_BOUND ( 'NONE', #94820, .T. ) ;
#86393=CIRCLE ( 'NONE', #101172, 0.1000000000000002554 ) ;
#86395=ORIENTED_EDGE ( 'NONE', *, *, #1907, .T. ) ;
#86396=CARTESIAN_POINT ( 'NONE',  ( -3.100000000000028511, 2.500000000000000000, -0.4464101615137782142 ) ) ;
#86397=FACE_OUTER_BOUND ( 'NONE', #108564, .T. ) ;
#86398=CARTESIAN_POINT ( 'NONE',  ( -7.950000000000012612, 12.50000000000000000, -2.165063509461101710 ) ) ;
#86399=LINE ( 'NONE', #46475, #29494 ) ;
#86400=EDGE_LOOP ( 'NONE', ( #109664, #107687 ) ) ;
#86401=DIRECTION ( 'NONE',  ( 0.000000000000000000, 0.000000000000000000, -1.000000000000000000 ) ) ;
#86402=EDGE_CURVE ( 'NONE', #6482, #84545, #39563, .T. ) ;
#86403=ORIENTED_EDGE ( 'NONE', *, *, #47928, .T. ) ;
#86404=EDGE_LOOP ( 'NONE', ( #44660, #35169, #48107, #17368 ) ) ;
#86405=AXIS2_PLACEMENT_3D ( 'NONE', #46419, #55606, #95539 ) ;
#86406=ORIENTED_EDGE ( 'NONE', *, *, #95401, .F. ) ;
#86407=CIRCLE ( 'NONE', #84365, 0.09999999999999982514 ) ;
#86408=CARTESIAN_POINT ( 'NONE',  ( -9.550000000000006040, 12.50000000000000000, 2.165063509461097713 ) ) ;
#86409=FACE_BOUND ( 'NONE', #109021, .T. ) ;
#86410=DIRECTION ( 'NONE',  ( -4.274815082592931898E-19, -0.9999939076577903929, -0.003490651415223739937 ) ) ;
#86411=DIRECTION ( 'NONE',  ( 0.000000000000000000, -0.000000000000000000, 1.000000000000000000 ) ) ;
#86412=CARTESIAN_POINT ( 'NONE',  ( -4.800000000000028244, 2.500000000000000000, -3.983716857408426293 ) ) ;
#86413=EDGE_CURVE ( 'NONE', #119463, #116333, #80104, .T. ) ;
#86414=AXIS2_PLACEMENT_3D ( 'NONE', #63878, #103803, #65137 ) ;
#86416=CONICAL_SURFACE ( 'NONE', #55135, 0.1000000000000000472, 0.003490658503988666988 ) ;
#86417=AXIS2_PLACEMENT_3D ( 'NONE', #83611, #31930, #114974 ) ;
#86418=CONICAL_SURFACE ( 'NONE', #96885, 0.1000000000000002554, 0.003490658503988666988 ) ;
#86419=EDGE_LOOP ( 'NONE', ( #90006, #127590 ) ) ;
#86420=CARTESIAN_POINT ( 'NONE',  ( -6.850000000000017408, 12.50000000000000000, -6.906693963081115051 ) ) ;
#86421=CARTESIAN_POINT ( 'NONE',  ( -7.300000000000013145, 2.500000000000000000, 3.983716857408420076 ) ) ;
#86422=DIRECTION ( 'NONE',  ( -0.000000000000000000, 1.000000000000000000, -0.000000000000000000 ) ) ;
#86423=CARTESIAN_POINT ( 'NONE',  ( -4.600000000000028955, 2.500000000000000000, -4.230127018922201998 ) ) ;
#86424=ORIENTED_EDGE ( 'NONE', *, *, #55054, .T. ) ;
#86425=AXIS2_PLACEMENT_3D ( 'NONE', #22982, #62899, #102802 ) ;
#86426=DIRECTION ( 'NONE',  ( 0.000000000000000000, -0.000000000000000000, 1.000000000000000000 ) ) ;
#86427=CIRCLE ( 'NONE', #30022, 0.1000000000000002554 ) ;
#86428=CONICAL_SURFACE ( 'NONE', #40498, 0.1000000000000002554, 0.003490658503988666988 ) ;
#86429=FACE_OUTER_BOUND ( 'NONE', #64924, .T. ) ;
#86430=AXIS2_PLACEMENT_3D ( 'NONE', #35165, #126760, #4363 ) ;
#86431=ORIENTED_EDGE ( 'NONE', *, *, #93162, .T. ) ;
#86432=CONICAL_SURFACE ( 'NONE', #115677, 0.1000000000000002554, 0.003490658503988666988 ) ;
#86433=CARTESIAN_POINT ( 'NONE',  ( -9.150000000000009237, 12.50000000000000000, -6.495190528383297135 ) ) ;
#86434=CARTESIAN_POINT ( 'NONE',  ( 11.24999999999994493, 12.50000000000000000, 6.560283801567334372 ) ) ;
#86435=FACE_BOUND ( 'NONE', #2317, .T. ) ;
#86436=DIRECTION ( 'NONE',  ( -0.000000000000000000, 1.000000000000000000, -0.000000000000000000 ) ) ;
#86437=ORIENTED_EDGE ( 'NONE', *, *, #2270, .T. ) ;
#86438=FACE_OUTER_BOUND ( 'NONE', #95071, .T. ) ;
#86439=DIRECTION ( 'NONE',  ( 0.000000000000000000, -0.9999939076577903929, 0.003490651415223739937 ) ) ;
#86441=VERTEX_POINT ( 'NONE', #48718 ) ;
#86443=AXIS2_PLACEMENT_3D ( 'NONE', #86421, #116527, #126360 ) ;
#86444=EDGE_LOOP ( 'NONE', ( #10023, #125968 ) ) ;
#86446=CARTESIAN_POINT ( 'NONE',  ( -9.800000000000004263, 2.500000000000000000, 3.983716857408420076 ) ) ;
#86448=CARTESIAN_POINT ( 'NONE',  ( -1.900000000000034550, 2.500000000000000000, 4.676537180435972552 ) ) ;
#86449=CARTESIAN_POINT ( 'NONE',  ( 11.24999999999994493, 2.500000000000000000, 6.495190528383297135 ) ) ;
#86450=AXIS2_PLACEMENT_3D ( 'NONE', #21372, #22039, #29915 ) ;
#86451=VECTOR ( 'NONE', #36881, 1000.000000000000000 ) ;
#86452=EDGE_CURVE ( 'NONE', #82955, #65404, #118729, .T. ) ;
#86453=CONICAL_SURFACE ( 'NONE', #32113, 0.1000000000000002554, 0.003490658503988666988 ) ;
#86454=ORIENTED_EDGE ( 'NONE', *, *, #70778, .T. ) ;
#86455=DIRECTION ( 'NONE',  ( 0.000000000000000000, -0.9999939076577903929, 0.003490651415223739937 ) ) ;
#86456=CARTESIAN_POINT ( 'NONE',  ( -3.550000000000027356, 2.500000000000000000, -2.511473670974877948 ) ) ;
#86457=DIRECTION ( 'NONE',  ( -4.274815082592931898E-19, -0.9999939076577903929, -0.003490651415223739937 ) ) ;
#86458=DIRECTION ( 'NONE',  ( 0.000000000000000000, -0.9999939076577903929, 0.003490651415223739937 ) ) ;
#86459=VERTEX_POINT ( 'NONE', #9426 ) ;
#86460=EDGE_CURVE ( 'NONE', #62381, #12101, #14331, .T. ) ;
#86461=DIRECTION ( 'NONE',  ( -0.000000000000000000, 1.000000000000000000, -0.000000000000000000 ) ) ;
#86462=EDGE_LOOP ( 'NONE', ( #6945, #91167 ) ) ;
#86463=CIRCLE ( 'NONE', #55180, 0.06509327318403745899 ) ;
#86464=ADVANCED_FACE ( 'NONE', ( #119366 ), #29709, .T. ) ;
#86465=DIRECTION ( 'NONE',  ( -0.000000000000000000, 1.000000000000000000, -0.000000000000000000 ) ) ;
#86466=FACE_OUTER_BOUND ( 'NONE', #72366, .T. ) ;
#86467=ORIENTED_EDGE ( 'NONE', *, *, #83534, .F. ) ;
#86468=AXIS2_PLACEMENT_3D ( 'NONE', #31770, #30497, #102439 ) ;
#86469=CARTESIAN_POINT ( 'NONE',  ( -4.150000000000025224, 2.500000000000000000, -1.472243186433550122 ) ) ;
#86470=CARTESIAN_POINT ( 'NONE',  ( 87.50000000000000000, -4.424430252271037922, -6.079088403633667426 ) ) ;
#86471=VECTOR ( 'NONE', #42305, 1000.000000000000000 ) ;
#86472=CARTESIAN_POINT ( 'NONE',  ( 9.999999999999948486, 12.50000000000000000, 4.395220292106234439 ) ) ;
#86473=DIRECTION ( 'NONE',  ( -4.274815082592931898E-19, -0.9999939076577903929, -0.003490651415223739937 ) ) ;
#86474=ORIENTED_EDGE ( 'NONE', *, *, #51343, .T. ) ;
#86475=ADVANCED_FACE ( 'NONE', ( #59846 ), #120962, .T. ) ;
#86476=CARTESIAN_POINT ( 'NONE',  ( 5.849999999999933031, 2.500000000000000000, 7.188010851410848723 ) ) ;
#86477=DIRECTION ( 'NONE',  ( 0.000000000000000000, 0.000000000000000000, 1.000000000000000000 ) ) ;
#86479=DIRECTION ( 'NONE',  ( -0.000000000000000000, 1.000000000000000000, -0.000000000000000000 ) ) ;
#86480=EDGE_CURVE ( 'NONE', #47772, #86058, #125011, .T. ) ;
#86481=DIRECTION ( 'NONE',  ( 0.000000000000000000, -0.9999939076577903929, 0.003490651415223739937 ) ) ;
#86482=ORIENTED_EDGE ( 'NONE', *, *, #96524, .T. ) ;
#86483=VERTEX_POINT ( 'NONE', #26173 ) ;
#86484=CARTESIAN_POINT ( 'NONE',  ( 0.5999999999999547917, 2.500000000000000000, 3.983716857408420076 ) ) ;
#86485=VECTOR ( 'NONE', #25731, 1000.000000000000000 ) ;
#86486=ORIENTED_EDGE ( 'NONE', *, *, #48875, .F. ) ;
#86487=DIRECTION ( 'NONE',  ( 0.000000000000000000, 0.000000000000000000, -1.000000000000000000 ) ) ;
#86488=ORIENTED_EDGE ( 'NONE', *, *, #3443, .T. ) ;
#86489=ORIENTED_EDGE ( 'NONE', *, *, #127819, .F. ) ;
#86490=ORIENTED_EDGE ( 'NONE', *, *, #62602, .F. ) ;
#86491=CIRCLE ( 'NONE', #25957, 0.06509327318403745899 ) ;
#86492=DIRECTION ( 'NONE',  ( -0.000000000000000000, -1.000000000000000000, -0.000000000000000000 ) ) ;
#86493=VECTOR ( 'NONE', #128491, 1000.000000000000000 ) ;
#86494=DIRECTION ( 'NONE',  ( 0.000000000000000000, 0.000000000000000000, -1.000000000000000000 ) ) ;
#86495=DIRECTION ( 'NONE',  ( 0.000000000000000000, -0.000000000000000000, 1.000000000000000000 ) ) ;
#86496=DIRECTION ( 'NONE',  ( 0.000000000000000000, 0.000000000000000000, 1.000000000000000000 ) ) ;
#86497=DIRECTION ( 'NONE',  ( -4.274815082592931898E-19, -0.9999939076577903929, -0.003490651415223739937 ) ) ;
#86498=CARTESIAN_POINT ( 'NONE',  ( -3.750000000000027978, 12.50000000000000000, 7.188010851410848723 ) ) ;
#86500=DIRECTION ( 'NONE',  ( 0.000000000000000000, -0.000000000000000000, 1.000000000000000000 ) ) ;
#86502=ORIENTED_EDGE ( 'NONE', *, *, #1956, .T. ) ;
#86503=ORIENTED_EDGE ( 'NONE', *, *, #103667, .T. ) ;
#86504=EDGE_LOOP ( 'NONE', ( #51230, #53004 ) ) ;
#86505=DIRECTION ( 'NONE',  ( 0.000000000000000000, 0.000000000000000000, -1.000000000000000000 ) ) ;
#86506=CONICAL_SURFACE ( 'NONE', #46814, 0.09999999999999982514, 0.003490658503988666988 ) ;
#86507=ORIENTED_EDGE ( 'NONE', *, *, #65788, .F. ) ;
#86508=VERTEX_POINT ( 'NONE', #85084 ) ;
#86509=CONICAL_SURFACE ( 'NONE', #4926, 0.1000000000000002554, 0.003490658503988666988 ) ;
#86510=DIRECTION ( 'NONE',  ( 0.000000000000000000, 0.000000000000000000, 1.000000000000000000 ) ) ;
#86511=AXIS2_PLACEMENT_3D ( 'NONE', #84120, #24567, #54031 ) ;
#86512=LINE ( 'NONE', #115981, #94239 ) ;
#86513=DIRECTION ( 'NONE',  ( 0.000000000000000000, 1.000000000000000000, 0.000000000000000000 ) ) ;
#86514=CARTESIAN_POINT ( 'NONE',  ( -6.250000000000021316, 2.500000000000000000, -1.572243186433550211 ) ) ;
#86515=AXIS2_PLACEMENT_3D ( 'NONE', #2290, #33084, #3596 ) ;
#86516=VECTOR ( 'NONE', #19750, 1000.000000000000000 ) ;
#86517=ADVANCED_FACE ( 'NONE', ( #115834 ), #125641, .T. ) ;
#86518=FACE_OUTER_BOUND ( 'NONE', #9379, .T. ) ;
#86519=EDGE_LOOP ( 'NONE', ( #114944, #113191 ) ) ;
#86520=ADVANCED_FACE ( 'NONE', ( #75905 ), #43616, .T. ) ;
#86521=EDGE_CURVE ( 'NONE', #90795, #121936, #14398, .T. ) ;
#86522=DIRECTION ( 'NONE',  ( 0.000000000000000000, -0.9999939076577903929, 0.003490651415223739937 ) ) ;
#86523=EDGE_CURVE ( 'NONE', #57299, #123681, #97970, .T. ) ;
#86524=AXIS2_PLACEMENT_3D ( 'NONE', #54838, #75771, #23457 ) ;
#86525=CONICAL_SURFACE ( 'NONE', #40595, 0.1000000000000000472, 0.003490658503988666988 ) ;
#86526=VERTEX_POINT ( 'NONE', #66084 ) ;
#86527=DIRECTION ( 'NONE',  ( 0.000000000000000000, 1.000000000000000000, 0.000000000000000000 ) ) ;
#86528=AXIS2_PLACEMENT_3D ( 'NONE', #112702, #102238, #101591 ) ;
#86529=ORIENTED_EDGE ( 'NONE', *, *, #59793, .F. ) ;
#86530=DIRECTION ( 'NONE',  ( 0.000000000000000000, 0.000000000000000000, 1.000000000000000000 ) ) ;
#86531=EDGE_CURVE ( 'NONE', #20260, #38135, #41564, .T. ) ;
#86532=ORIENTED_EDGE ( 'NONE', *, *, #62292, .F. ) ;
#86533=VERTEX_POINT ( 'NONE', #73983 ) ;
#86534=DIRECTION ( 'NONE',  ( 0.000000000000000000, -0.000000000000000000, 1.000000000000000000 ) ) ;
#86535=DIRECTION ( 'NONE',  ( -4.274815082592931898E-19, -0.9999939076577903929, -0.003490651415223739937 ) ) ;
#86536=EDGE_CURVE ( 'NONE', #58995, #105130, #95558, .T. ) ;
#86537=EDGE_CURVE ( 'NONE', #53182, #43603, #123115, .T. ) ;
#86538=CARTESIAN_POINT ( 'NONE',  ( 14.14999999999989733, 2.500000000000000000, 1.372243186433545370 ) ) ;
#86539=CARTESIAN_POINT ( 'NONE',  ( 1.849999999999951017, 2.500000000000000000, -6.048780366869526581 ) ) ;
#86540=CARTESIAN_POINT ( 'NONE',  ( 1.249999999999986899, 12.50000000000000000, 6.560283801567334372 ) ) ;
#86541=ORIENTED_EDGE ( 'NONE', *, *, #40879, .T. ) ;
#86542=CARTESIAN_POINT ( 'NONE',  ( -9.800000000000004263, 12.50000000000000000, 3.918623584224382839 ) ) ;
#86543=CARTESIAN_POINT ( 'NONE',  ( 12.49999999999990585, 2.500000000000000000, 3.637306695894644726 ) ) ;
#86545=DIRECTION ( 'NONE',  ( 0.000000000000000000, 1.000000000000000000, 0.000000000000000000 ) ) ;
#86546=DIRECTION ( 'NONE',  ( 0.000000000000000000, 0.000000000000000000, 1.000000000000000000 ) ) ;
#86547=AXIS2_PLACEMENT_3D ( 'NONE', #18106, #125488, #55469 ) ;
#86548=DIRECTION ( 'NONE',  ( 0.000000000000000000, 0.000000000000000000, -1.000000000000000000 ) ) ;
#86549=ORIENTED_EDGE ( 'NONE', *, *, #5055, .T. ) ;
#86550=ORIENTED_EDGE ( 'NONE', *, *, #84116, .F. ) ;
#86551=DIRECTION ( 'NONE',  ( 0.000000000000000000, 0.000000000000000000, 1.000000000000000000 ) ) ;
#86552=EDGE_LOOP ( 'NONE', ( #41742, #52168, #128488, #95316 ) ) ;
#86553=CIRCLE ( 'NONE', #42671, 0.1000000000000002554 ) ;
#86554=CARTESIAN_POINT ( 'NONE',  ( -8.150000000000012790, 2.500000000000000000, 2.511473670974873507 ) ) ;
#86555=FACE_OUTER_BOUND ( 'NONE', #61662, .T. ) ;
#86556=CIRCLE ( 'NONE', #44812, 0.1000000000000002554 ) ;
#86557=ORIENTED_EDGE ( 'NONE', *, *, #112788, .F. ) ;
#86560=CARTESIAN_POINT ( 'NONE',  ( 7.699999999999925571, 2.500000000000000000, -4.676537180435978769 ) ) ;
#86562=ORIENTED_EDGE ( 'NONE', *, *, #92411, .T. ) ;
#86563=AXIS2_PLACEMENT_3D ( 'NONE', #65793, #105731, #27802 ) ;
#86564=CARTESIAN_POINT ( 'NONE',  ( 16.56576425165007649, -1.499999999999997113, -6.084390597445788806 ) ) ;
#86565=CARTESIAN_POINT ( 'NONE',  ( 8.099999999999921485, 12.50000000000000000, 0.2813168883297361700 ) ) ;
#86566=VERTEX_POINT ( 'NONE', #113251 ) ;
#86568=DIRECTION ( 'NONE',  ( 0.000000000000000000, 1.000000000000000000, 0.000000000000000000 ) ) ;
#86569=CARTESIAN_POINT ( 'NONE',  ( -13.09999999999999076, 2.500000000000000000, 4.676537180435972552 ) ) ;
#86570=EDGE_CURVE ( 'NONE', #83172, #27784, #55629, .T. ) ;
#86571=ORIENTED_EDGE ( 'NONE', *, *, #87093, .F. ) ;
#86572=CIRCLE ( 'NONE', #30166, 0.1000000000000002554 ) ;
#86573=VECTOR ( 'NONE', #23515, 1000.000000000000000 ) ;
#86574=CIRCLE ( 'NONE', #5000, 0.1000000000000002554 ) ;
#86575=CARTESIAN_POINT ( 'NONE',  ( -11.64999999999999858, 12.50000000000000000, -1.472243186433546125 ) ) ;
#86576=CONICAL_SURFACE ( 'NONE', #67705, 0.1000000000000000472, 0.003490658503988666988 ) ;
#86577=ORIENTED_EDGE ( 'NONE', *, *, #15215, .T. ) ;
#86578=CARTESIAN_POINT ( 'NONE',  ( 9.399999999999915090, 2.500000000000000000, 4.083716857408421497 ) ) ;
#86579=CARTESIAN_POINT ( 'NONE',  ( -4.350000000000023626, 2.500000000000000000, -2.511473670974877948 ) ) ;
#86580=FACE_OUTER_BOUND ( 'NONE', #60434, .T. ) ;
#86581=AXIS2_PLACEMENT_3D ( 'NONE', #80332, #40419, #107848 ) ;
#86582=EDGE_LOOP ( 'NONE', ( #48162, #53245, #114823, #50219 ) ) ;
#86583=CARTESIAN_POINT ( 'NONE',  ( 10.39999999999990976, 2.500000000000000000, -4.430127018922202176 ) ) ;
#86584=CARTESIAN_POINT ( 'NONE',  ( -2.900000000000029221, 2.500000000000000000, -2.276824562219559311E-15 ) ) ;
#86585=ORIENTED_EDGE ( 'NONE', *, *, #33068, .T. ) ;
#86586=ORIENTED_EDGE ( 'NONE', *, *, #73435, .T. ) ;
#86587=CARTESIAN_POINT ( 'NONE',  ( 7.899999999999924860, 12.50000000000000000, 3.637306695894644726 ) ) ;
#86588=CIRCLE ( 'NONE', #17637, 0.1000000000000002554 ) ;
#86589=VERTEX_POINT ( 'NONE', #114532 ) ;
#86590=CARTESIAN_POINT ( 'NONE',  ( -1.250000000000035749, 2.500000000000000000, -7.188010851410854052 ) ) ;
#86591=CARTESIAN_POINT ( 'NONE',  ( 3.749999999999940492, 12.50000000000000000, 2.792790559304612064 ) ) ;
#86592=AXIS2_PLACEMENT_3D ( 'NONE', #105203, #57406, #24722 ) ;
#86593=AXIS2_PLACEMENT_3D ( 'NONE', #70429, #80256, #18095 ) ;
#86594=AXIS2_PLACEMENT_3D ( 'NONE', #111760, #31280, #50916 ) ;
#86595=VERTEX_POINT ( 'NONE', #75261 ) ;
#86596=ORIENTED_EDGE ( 'NONE', *, *, #58870, .T. ) ;
#86597=DIRECTION ( 'NONE',  ( 0.000000000000000000, 0.000000000000000000, -1.000000000000000000 ) ) ;
#86598=CARTESIAN_POINT ( 'NONE',  ( 1.849999999999950573, 2.500000000000000000, -1.918653347947326004 ) ) ;
#86600=FACE_OUTER_BOUND ( 'NONE', #126521, .T. ) ;
#86601=AXIS2_PLACEMENT_3D ( 'NONE', #36852, #129113, #29592 ) ;
#86603=VECTOR ( 'NONE', #92810, 1000.000000000000000 ) ;
#86604=CIRCLE ( 'NONE', #115853, 0.06509327318403745899 ) ;
#86605=DIRECTION ( 'NONE',  ( 0.000000000000000000, 0.000000000000000000, 1.000000000000000000 ) ) ;
#86606=CARTESIAN_POINT ( 'NONE',  ( 7.699999999999922018, 2.500000000000000000, 0.2464101615137735679 ) ) ;
#86607=CARTESIAN_POINT ( 'NONE',  ( 12.94999999999989981, 12.50000000000000000, -2.099970236277064473 ) ) ;
#86608=FACE_OUTER_BOUND ( 'NONE', #83234, .T. ) ;
#86609=AXIS2_PLACEMENT_3D ( 'NONE', #7018, #7668, #29273 ) ;
#86611=CIRCLE ( 'NONE', #113733, 0.06509327318403745899 ) ;
#86613=VERTEX_POINT ( 'NONE', #34727 ) ;
#86614=VERTEX_POINT ( 'NONE', #63526 ) ;
#86615=EDGE_LOOP ( 'NONE', ( #20869, #91390, #37673, #16698 ) ) ;
#86617=DIRECTION ( 'NONE',  ( 0.000000000000000000, 0.000000000000000000, -1.000000000000000000 ) ) ;
#86618=CARTESIAN_POINT ( 'NONE',  ( 11.04999999999990656, 12.50000000000000000, -6.083687093685488989 ) ) ;
#86619=CONICAL_SURFACE ( 'NONE', #30217, 0.1000000000000002554, 0.003490658503988666988 ) ;
#86620=FACE_OUTER_BOUND ( 'NONE', #75064, .T. ) ;
#86621=ORIENTED_EDGE ( 'NONE', *, *, #57183, .T. ) ;
#86622=EDGE_CURVE ( 'NONE', #95311, #56692, #5863, .T. ) ;
#86623=FACE_BOUND ( 'NONE', #27507, .T. ) ;
#86624=ADVANCED_FACE ( 'NONE', ( #15682 ), #104327, .T. ) ;
#86625=LINE ( 'NONE', #35609, #18634 ) ;
#86626=DIRECTION ( 'NONE',  ( 0.000000000000000000, 0.000000000000000000, 1.000000000000000000 ) ) ;
#86627=DIRECTION ( 'NONE',  ( 0.000000000000000000, 0.000000000000000000, -1.000000000000000000 ) ) ;
#86628=CARTESIAN_POINT ( 'NONE',  ( -10.60000000000000320, 2.500000000000000000, -3.983716857408421852 ) ) ;
#86629=CARTESIAN_POINT ( 'NONE',  ( 3.749999999999976907, 2.500000000000000000, 2.265063509461097357 ) ) ;
#86630=EDGE_CURVE ( 'NONE', #85856, #6770, #3942, .T. ) ;
#86631=DIRECTION ( 'NONE',  ( 0.000000000000000000, 0.000000000000000000, 1.000000000000000000 ) ) ;
#86632=EDGE_CURVE ( 'NONE', #32010, #54474, #54166, .T. ) ;
#86633=VERTEX_POINT ( 'NONE', #113915 ) ;
#86634=DIRECTION ( 'NONE',  ( 0.000000000000000000, 0.000000000000000000, 1.000000000000000000 ) ) ;
#86635=ADVANCED_FACE ( 'NONE', ( #54337 ), #118995, .T. ) ;
#86636=DIRECTION ( 'NONE',  ( -0.000000000000000000, -1.000000000000000000, -0.000000000000000000 ) ) ;
#86638=EDGE_CURVE ( 'NONE', #29908, #32550, #14426, .T. ) ;
#86639=CIRCLE ( 'NONE', #101320, 0.06509327318403745899 ) ;
#86640=CARTESIAN_POINT ( 'NONE',  ( -8.550000000000011369, 2.500000000000000000, -2.511473670974877948 ) ) ;
#86641=ORIENTED_EDGE ( 'NONE', *, *, #93610, .F. ) ;
#86642=ORIENTED_EDGE ( 'NONE', *, *, #83556, .T. ) ;
#86643=EDGE_LOOP ( 'NONE', ( #73095, #6235 ) ) ;
#86644=ORIENTED_EDGE ( 'NONE', *, *, #102482, .T. ) ;
#86645=CARTESIAN_POINT ( 'NONE',  ( 9.549999999999915445, 12.50000000000000000, 6.495190528383297135 ) ) ;
#86646=CARTESIAN_POINT ( 'NONE',  ( 14.19999999999989626, 2.500000000000000000, -0.1000000000000022815 ) ) ;
#86647=ORIENTED_EDGE ( 'NONE', *, *, #118973, .F. ) ;
#86649=EDGE_CURVE ( 'NONE', #83282, #96180, #66754, .T. ) ;
#86650=ORIENTED_EDGE ( 'NONE', *, *, #73753, .F. ) ;
#86651=DIRECTION ( 'NONE',  ( 0.000000000000000000, 0.000000000000000000, 1.000000000000000000 ) ) ;
#86652=AXIS2_PLACEMENT_3D ( 'NONE', #33819, #73733, #16092 ) ;
#86653=AXIS2_PLACEMENT_3D ( 'NONE', #89022, #20271, #41226 ) ;
#86654=CARTESIAN_POINT ( 'NONE',  ( 10.30524027341030369, -2.500000000000510703, 9.130939513284465292 ) ) ;
#86655=DIRECTION ( 'NONE',  ( 0.000000000000000000, 1.000000000000000000, 0.000000000000000000 ) ) ;
#86656=DIRECTION ( 'NONE',  ( 0.000000000000000000, 1.000000000000000000, 0.000000000000000000 ) ) ;
#86657=DIRECTION ( 'NONE',  ( 0.000000000000000000, 1.000000000000000000, 0.000000000000000000 ) ) ;
#86658=ORIENTED_EDGE ( 'NONE', *, *, #55364, .F. ) ;
#86659=EDGE_LOOP ( 'NONE', ( #32450, #45524 ) ) ;
#86660=CIRCLE ( 'NONE', #26034, 0.06509327318403745899 ) ;
#86661=ORIENTED_EDGE ( 'NONE', *, *, #17830, .F. ) ;
#86662=ORIENTED_EDGE ( 'NONE', *, *, #97709, .F. ) ;
#86663=AXIS2_PLACEMENT_3D ( 'NONE', #68096, #107387, #3 ) ;
#86664=DIRECTION ( 'NONE',  ( 0.000000000000000000, 1.000000000000000000, 0.000000000000000000 ) ) ;
#86665=ORIENTED_EDGE ( 'NONE', *, *, #33329, .F. ) ;
#86666=EDGE_LOOP ( 'NONE', ( #111244, #81725, #77207, #106152 ) ) ;
#86667=CARTESIAN_POINT ( 'NONE',  ( 4.399999999999939071, 12.50000000000000000, -0.3464101615137782364 ) ) ;
#86668=CARTESIAN_POINT ( 'NONE',  ( -3.150000000000029665, 2.500000000000000000, 6.841600689897072485 ) ) ;
#86669=AXIS2_PLACEMENT_3D ( 'NONE', #54711, #40593, #101421 ) ;
#86670=CARTESIAN_POINT ( 'NONE',  ( -7.050000000000013145, 12.50000000000000000, 2.099970236277060032 ) ) ;
#86671=CIRCLE ( 'NONE', #30263, 0.09999999999999999167 ) ;
#86672=DIRECTION ( 'NONE',  ( 0.000000000000000000, -0.000000000000000000, 1.000000000000000000 ) ) ;
#86673=ADVANCED_FACE ( 'NONE', ( #116467 ), #98761, .T. ) ;
#86674=FACE_OUTER_BOUND ( 'NONE', #93090, .T. ) ;
#86675=CIRCLE ( 'NONE', #15559, 0.1000000000000002554 ) ;
#86676=ADVANCED_FACE ( 'NONE', ( #9100 ), #121052, .T. ) ;
#86677=VERTEX_POINT ( 'NONE', #26815 ) ;
#86678=EDGE_CURVE ( 'NONE', #28644, #63269, #49695, .T. ) ;
#86679=CIRCLE ( 'NONE', #61571, 0.06509327318403745899 ) ;
#86680=FACE_OUTER_BOUND ( 'NONE', #83797, .T. ) ;
#86681=ORIENTED_EDGE ( 'NONE', *, *, #927, .F. ) ;
#86683=EDGE_CURVE ( 'NONE', #34661, #46223, #47750, .T. ) ;
#86684=VERTEX_POINT ( 'NONE', #27439 ) ;
#86685=DIRECTION ( 'NONE',  ( 0.000000000000000000, 1.000000000000000000, 0.000000000000000000 ) ) ;
#86686=CARTESIAN_POINT ( 'NONE',  ( 10.59999999999991260, 2.500000000000000000, 0.2464101615137735679 ) ) ;
#86687=ORIENTED_EDGE ( 'NONE', *, *, #93143, .F. ) ;
#86688=CARTESIAN_POINT ( 'NONE',  ( -6.850000000000013856, 12.50000000000000000, 2.511473670974873507 ) ) ;
#86689=ADVANCED_FACE ( 'NONE', ( #128252 ), #41662, .T. ) ;
#86690=CARTESIAN_POINT ( 'NONE',  ( -4.350000000000027178, 2.500000000000000000, -6.841600689897077814 ) ) ;
#86691=ORIENTED_EDGE ( 'NONE', *, *, #76607, .F. ) ;
#86692=ADVANCED_FACE ( 'NONE', ( #38592 ), #127327, .T. ) ;
#86693=EDGE_CURVE ( 'NONE', #90873, #118431, #116835, .T. ) ;
#86694=EDGE_CURVE ( 'NONE', #92950, #32930, #16566, .T. ) ;
#86695=VECTOR ( 'NONE', #128902, 1000.000000000000000 ) ;
#86696=VECTOR ( 'NONE', #23931, 1000.000000000000000 ) ;
#86697=FACE_OUTER_BOUND ( 'NONE', #92760, .T. ) ;
#86698=ORIENTED_EDGE ( 'NONE', *, *, #80658, .T. ) ;
#86699=CONICAL_SURFACE ( 'NONE', #69985, 0.1000000000000002554, 0.003490658503988666988 ) ;
#86700=VERTEX_POINT ( 'NONE', #47114 ) ;
#86701=DIRECTION ( 'NONE',  ( 0.000000000000000000, 0.000000000000000000, 1.000000000000000000 ) ) ;
#86702=CARTESIAN_POINT ( 'NONE',  ( 8.149999999999923972, 12.50000000000000000, -6.776507416713039689 ) ) ;
#86704=CARTESIAN_POINT ( 'NONE',  ( 9.349999999999916156, 2.500000000000000000, -2.511473670974877948 ) ) ;
#86705=EDGE_CURVE ( 'NONE', #125180, #93363, #64616, .T. ) ;
#86706=CONICAL_SURFACE ( 'NONE', #32453, 0.1000000000000002554, 0.003490658503988666988 ) ;
#86707=DIRECTION ( 'NONE',  ( 0.000000000000000000, 0.000000000000000000, -1.000000000000000000 ) ) ;
#86708=VECTOR ( 'NONE', #56833, 1000.000000000000000 ) ;
#86709=CONICAL_SURFACE ( 'NONE', #36555, 0.09999999999999999167, 0.003490658503988666988 ) ;
#86710=PLANE ( 'NONE',  #8967 ) ;
#86711=CIRCLE ( 'NONE', #109708, 0.06509327318403745899 ) ;
#86712=VERTEX_POINT ( 'NONE', #68020 ) ;
#86713=AXIS2_PLACEMENT_3D ( 'NONE', #124205, #73804, #33887 ) ;
#86714=CARTESIAN_POINT ( 'NONE',  ( -13.14999999999999147, 12.50000000000000000, -2.511473670974875727 ) ) ;
#86715=AXIS2_PLACEMENT_3D ( 'NONE', #76493, #93546, #64722 ) ;
#86716=ORIENTED_EDGE ( 'NONE', *, *, #127903, .F. ) ;
#86717=AXIS2_PLACEMENT_3D ( 'NONE', #105861, #16161, #46284 ) ;
#86718=CARTESIAN_POINT ( 'NONE',  ( -13.29999999999998828, 2.500000000000000000, 4.330127018922196314 ) ) ;
#86719=DIRECTION ( 'NONE',  ( -0.000000000000000000, 1.000000000000000000, -0.000000000000000000 ) ) ;
#86720=ADVANCED_FACE ( 'NONE', ( #119063 ), #123216, .T. ) ;
#86721=DIRECTION ( 'NONE',  ( 0.000000000000000000, 0.000000000000000000, 1.000000000000000000 ) ) ;
#86722=DIRECTION ( 'NONE',  ( 0.000000000000000000, -0.9999939076577903929, 0.003490651415223739937 ) ) ;
#86723=CARTESIAN_POINT ( 'NONE',  ( -0.4000000000000404898, 12.50000000000000000, 5.022947341949748790 ) ) ;
#86724=EDGE_LOOP ( 'NONE', ( #122202, #5692, #70722, #78074 ) ) ;
#86725=FACE_OUTER_BOUND ( 'NONE', #73058, .T. ) ;
#86726=CARTESIAN_POINT ( 'NONE',  ( -6.900000000000019007, 2.500000000000000000, -4.083716857408426826 ) ) ;
#86727=CIRCLE ( 'NONE', #5247, 10.00000000000000000 ) ;
#86728=ORIENTED_EDGE ( 'NONE', *, *, #65101, .F. ) ;
#86729=CARTESIAN_POINT ( 'NONE',  ( 3.749999999999940492, 2.500000000000000000, 5.702370205355745014 ) ) ;
#86730=EDGE_CURVE ( 'NONE', #119380, #15697, #91814, .T. ) ;
#86731=EDGE_LOOP ( 'NONE', ( #40187, #6769, #58805, #71426 ) ) ;
#86732=VERTEX_POINT ( 'NONE', #109222 ) ;
#86733=CARTESIAN_POINT ( 'NONE',  ( -0.8500000000000395017, 2.500000000000000000, 2.165063509461097713 ) ) ;
#86734=ORIENTED_EDGE ( 'NONE', *, *, #90042, .T. ) ;
#86736=CARTESIAN_POINT ( 'NONE',  ( 2.699999999999947331, 2.500000000000000000, -0.3464101615137783474 ) ) ;
#86737=AXIS2_PLACEMENT_3D ( 'NONE', #103048, #43515, #52037 ) ;
#86738=DIRECTION ( 'NONE',  ( -0.000000000000000000, 1.000000000000000000, -0.000000000000000000 ) ) ;
#86739=ORIENTED_EDGE ( 'NONE', *, *, #104212, .F. ) ;
#86740=FACE_BOUND ( 'NONE', #33204, .T. ) ;
#86741=LINE ( 'NONE', #74999, #59945 ) ;
#86742=ORIENTED_EDGE ( 'NONE', *, *, #129403, .T. ) ;
#86743=CARTESIAN_POINT ( 'NONE',  ( -3.350000000000031619, 2.500000000000000000, -7.188010851410854052 ) ) ;
#86744=EDGE_CURVE ( 'NONE', #1738, #105627, #10333, .T. ) ;
#86745=PLANE ( 'NONE',  #13294 ) ;
#86746=EDGE_LOOP ( 'NONE', ( #68989, #88222 ) ) ;
#86747=VECTOR ( 'NONE', #17155, 1000.000000000000000 ) ;
#86748=ORIENTED_EDGE ( 'NONE', *, *, #45929, .T. ) ;
#86749=VERTEX_POINT ( 'NONE', #57576 ) ;
#86750=DIRECTION ( 'NONE',  ( -4.274815082592931898E-19, -0.9999939076577903929, -0.003490651415223739937 ) ) ;
#86751=LINE ( 'NONE', #16700, #26894 ) ;
#86752=DIRECTION ( 'NONE',  ( 0.000000000000000000, 0.000000000000000000, -1.000000000000000000 ) ) ;
#86753=FACE_BOUND ( 'NONE', #47525, .T. ) ;
#86754=ORIENTED_EDGE ( 'NONE', *, *, #112538, .T. ) ;
#86755=DIRECTION ( 'NONE',  ( 0.000000000000000000, 0.000000000000000000, -1.000000000000000000 ) ) ;
#86756=DIRECTION ( 'NONE',  ( -0.000000000000000000, -1.000000000000000000, -0.000000000000000000 ) ) ;
#86757=CARTESIAN_POINT ( 'NONE',  ( -14.99999999999998224, 12.50000000000000000, -0.7579135962115893799 ) ) ;
#86758=AXIS2_PLACEMENT_3D ( 'NONE', #1620, #81487, #42878 ) ;
#86759=DIRECTION ( 'NONE',  ( 0.000000000000000000, 1.000000000000000000, 0.000000000000000000 ) ) ;
#86760=DIRECTION ( 'NONE',  ( 0.000000000000000000, 1.000000000000000000, 0.000000000000000000 ) ) ;
#86761=PLANE ( 'NONE',  #128633 ) ;
#86762=FACE_OUTER_BOUND ( 'NONE', #44598, .T. ) ;
#86763=EDGE_CURVE ( 'NONE', #48547, #6862, #70888, .T. ) ;
#86764=ORIENTED_EDGE ( 'NONE', *, *, #116502, .T. ) ;
#86765=EDGE_LOOP ( 'NONE', ( #26628, #51862, #21210, #41850 ) ) ;
#86766=VERTEX_POINT ( 'NONE', #39243 ) ;
#86767=EDGE_LOOP ( 'NONE', ( #11435, #46461, #45315, #70380 ) ) ;
#86768=ORIENTED_EDGE ( 'NONE', *, *, #7625, .T. ) ;
#86769=DIRECTION ( 'NONE',  ( 0.000000000000000000, 0.000000000000000000, 1.000000000000000000 ) ) ;
#86770=CARTESIAN_POINT ( 'NONE',  ( -11.84999999999999609, 2.500000000000000000, 2.511473670974873507 ) ) ;
#86771=ORIENTED_EDGE ( 'NONE', *, *, #100378, .F. ) ;
#86772=FACE_BOUND ( 'NONE', #50381, .T. ) ;
#86773=AXIS2_PLACEMENT_3D ( 'NONE', #50446, #93596, #53671 ) ;
#86774=EDGE_CURVE ( 'NONE', #117651, #84736, #73028, .T. ) ;
#86775=CARTESIAN_POINT ( 'NONE',  ( 6.899999999999928413, 2.500000000000000000, -3.883716857408426648 ) ) ;
#86776=AXIS2_PLACEMENT_3D ( 'NONE', #129322, #21933, #91949 ) ;
#86777=CARTESIAN_POINT ( 'NONE',  ( 1.849999999999949685, 12.50000000000000000, 1.883746621131358934 ) ) ;
#86778=ADVANCED_FACE ( 'NONE', ( #20859 ), #125257, .T. ) ;
#86779=CIRCLE ( 'NONE', #124446, 0.06509327318403745899 ) ;
#86780=DIRECTION ( 'NONE',  ( 0.000000000000000000, 0.000000000000000000, -1.000000000000000000 ) ) ;
#86781=EDGE_CURVE ( 'NONE', #119766, #30225, #30703, .T. ) ;
#86782=PLANE ( 'NONE',  #19762 ) ;
#86783=ADVANCED_FACE ( 'NONE', ( #40523 ), #110525, .T. ) ;
#86784=CARTESIAN_POINT ( 'NONE',  ( 11.69999999999990514, 2.500000000000000000, -2.276824562219559311E-15 ) ) ;
#86785=ADVANCED_FACE ( 'NONE', ( #62089 ), #24911, .T. ) ;
#86786=ORIENTED_EDGE ( 'NONE', *, *, #19997, .F. ) ;
#86787=DIRECTION ( 'NONE',  ( 0.000000000000000000, 1.000000000000000000, 0.000000000000000000 ) ) ;
#86788=VERTEX_POINT ( 'NONE', #102629 ) ;
#86789=AXIS2_PLACEMENT_3D ( 'NONE', #40466, #81019, #90833 ) ;
#86790=AXIS2_PLACEMENT_3D ( 'NONE', #75411, #34228, #15187 ) ;
#86791=ORIENTED_EDGE ( 'NONE', *, *, #48209, .F. ) ;
#86792=ORIENTED_EDGE ( 'NONE', *, *, #110015, .F. ) ;
#86793=DIRECTION ( 'NONE',  ( 0.000000000000000000, 0.000000000000000000, -1.000000000000000000 ) ) ;
#86794=AXIS2_PLACEMENT_3D ( 'NONE', #126660, #16669, #97827 ) ;
#86795=DIRECTION ( 'NONE',  ( -4.274815082592931898E-19, -0.9999939076577903929, -0.003490651415223739937 ) ) ;
#86796=LINE ( 'NONE', #66506, #795 ) ;
#86797=ORIENTED_EDGE ( 'NONE', *, *, #5924, .T. ) ;
#86798=ADVANCED_FACE ( 'NONE', ( #11019 ), #1914, .T. ) ;
#86799=CARTESIAN_POINT ( 'NONE',  ( 4.599999999999938360, 2.500000000000000000, -2.276824562219559311E-15 ) ) ;
#86800=ADVANCED_FACE ( 'NONE', ( #12951 ), #26979, .T. ) ;
#86801=AXIS2_PLACEMENT_3D ( 'NONE', #112878, #52031, #114166 ) ;
#86802=CARTESIAN_POINT ( 'NONE',  ( 5.399999999999936406, 2.500000000000000000, -5.022947341949754119 ) ) ;
#86803=EDGE_CURVE ( 'NONE', #75566, #90750, #60445, .T. ) ;
#86804=DIRECTION ( 'NONE',  ( 0.000000000000000000, 1.000000000000000000, 0.000000000000000000 ) ) ;
#86806=DIRECTION ( 'NONE',  ( 0.000000000000000000, 0.000000000000000000, 1.000000000000000000 ) ) ;
#86807=DIRECTION ( 'NONE',  ( 0.000000000000000000, 1.000000000000000000, 0.000000000000000000 ) ) ;
#86808=VECTOR ( 'NONE', #47924, 1000.000000000000000 ) ;
#86810=CARTESIAN_POINT ( 'NONE',  ( -4.400000000000028777, 12.50000000000000000, -4.048810130592463530 ) ) ;
#86811=ORIENTED_EDGE ( 'NONE', *, *, #116555, .T. ) ;
#86812=CARTESIAN_POINT ( 'NONE',  ( -12.69999999999999218, 2.500000000000000000, -0.2464101615137741230 ) ) ;
#86813=ORIENTED_EDGE ( 'NONE', *, *, #39836, .T. ) ;
#86814=VERTEX_POINT ( 'NONE', #60162 ) ;
#86815=FACE_OUTER_BOUND ( 'NONE', #113048, .T. ) ;
#86816=DIRECTION ( 'NONE',  ( -0.000000000000000000, 1.000000000000000000, -0.000000000000000000 ) ) ;
#86817=DIRECTION ( 'NONE',  ( 0.000000000000000000, 1.000000000000000000, 0.000000000000000000 ) ) ;
#86818=VECTOR ( 'NONE', #97571, 1000.000000000000000 ) ;
#86819=ORIENTED_EDGE ( 'NONE', *, *, #67455, .F. ) ;
#86820=VERTEX_POINT ( 'NONE', #61447 ) ;
#86821=DIRECTION ( 'NONE',  ( 0.000000000000000000, 0.000000000000000000, -1.000000000000000000 ) ) ;
#86822=CARTESIAN_POINT ( 'NONE',  ( 48.81598501501260046, 3.619493961087981493, -4.312659849359727460 ) ) ;
#86823=DIRECTION ( 'NONE',  ( -4.274815082592931898E-19, -0.9999939076577903929, -0.003490651415223739937 ) ) ;
#86824=ORIENTED_EDGE ( 'NONE', *, *, #63037, .T. ) ;
#86825=ORIENTED_EDGE ( 'NONE', *, *, #55461, .T. ) ;
#86826=PLANE ( 'NONE',  #50288 ) ;
#86828=CIRCLE ( 'NONE', #61810, 0.06509327318403745899 ) ;
#86829=ORIENTED_EDGE ( 'NONE', *, *, #74363, .F. ) ;
#86830=CARTESIAN_POINT ( 'NONE',  ( 0.000000000000000000, 2.500000000000000000, 0.000000000000000000 ) ) ;
#86831=CIRCLE ( 'NONE', #1154, 0.06509327318403745899 ) ;
#86832=DIRECTION ( 'NONE',  ( 0.000000000000000000, -0.000000000000000000, 1.000000000000000000 ) ) ;
#86833=VERTEX_POINT ( 'NONE', #31341 ) ;
#86834=CARTESIAN_POINT ( 'NONE',  ( -12.49999999999999289, 12.50000000000000000, 5.022947341949748790 ) ) ;
#86835=PLANE ( 'NONE',  #12774 ) ;
#86836=DIRECTION ( 'NONE',  ( -4.274815082592931898E-19, -0.9999939076577903929, -0.003490651415223739937 ) ) ;
#86837=EDGE_CURVE ( 'NONE', #69080, #103801, #102001, .T. ) ;
#86838=DIRECTION ( 'NONE',  ( 0.000000000000000000, 1.000000000000000000, 0.000000000000000000 ) ) ;
#86839=ORIENTED_EDGE ( 'NONE', *, *, #115917, .T. ) ;
#86840=VECTOR ( 'NONE', #74671, 1000.000000000000000 ) ;
#86841=EDGE_CURVE ( 'NONE', #63043, #20499, #50981, .T. ) ;
#86842=DIRECTION ( 'NONE',  ( -0.000000000000000000, -1.000000000000000000, -0.000000000000000000 ) ) ;
#86843=DIRECTION ( 'NONE',  ( -0.000000000000000000, -1.000000000000000000, -0.000000000000000000 ) ) ;
#86844=AXIS2_PLACEMENT_3D ( 'NONE', #102556, #50901, #482 ) ;
#86845=EDGE_CURVE ( 'NONE', #114315, #23628, #121627, .T. ) ;
#86846=ORIENTED_EDGE ( 'NONE', *, *, #97437, .F. ) ;
#86847=EDGE_LOOP ( 'NONE', ( #27556, #14732, #57592, #5372 ) ) ;
#86849=DIRECTION ( 'NONE',  ( 0.000000000000000000, 1.000000000000000000, 0.000000000000000000 ) ) ;
#86850=DIRECTION ( 'NONE',  ( 0.000000000000000000, 0.000000000000000000, -1.000000000000000000 ) ) ;
#86851=CARTESIAN_POINT ( 'NONE',  ( -6.850000000000013856, 2.500000000000000000, 6.248780366869521430 ) ) ;
#86852=DIRECTION ( 'NONE',  ( 0.000000000000000000, 1.000000000000000000, 0.000000000000000000 ) ) ;
#86853=EDGE_CURVE ( 'NONE', #57270, #79310, #20711, .T. ) ;
#86854=CARTESIAN_POINT ( 'NONE',  ( -5.850000000000022737, 2.500000000000000000, -2.265063509461101798 ) ) ;
#86857=DIRECTION ( 'NONE',  ( -0.000000000000000000, 1.000000000000000000, -0.000000000000000000 ) ) ;
#86858=FACE_OUTER_BOUND ( 'NONE', #100925, .T. ) ;
#86859=PLANE ( 'NONE',  #98149 ) ;
#86860=VECTOR ( 'NONE', #93421, 1000.000000000000000 ) ;
#86861=VERTEX_POINT ( 'NONE', #71237 ) ;
#86862=DIRECTION ( 'NONE',  ( 0.000000000000000000, 1.000000000000000000, 0.000000000000000000 ) ) ;
#86863=VERTEX_POINT ( 'NONE', #72553 ) ;
#86864=DIRECTION ( 'NONE',  ( 0.000000000000000000, 1.000000000000000000, 0.000000000000000000 ) ) ;
#86865=CONICAL_SURFACE ( 'NONE', #59715, 0.1000000000000000056, 0.003490658503988666988 ) ;
#86866=ADVANCED_FACE ( 'NONE', ( #122298 ), #90887, .T. ) ;
#86867=DIRECTION ( 'NONE',  ( -0.000000000000000000, -1.000000000000000000, -0.000000000000000000 ) ) ;
#86868=CARTESIAN_POINT ( 'NONE',  ( 2.499999999999983569, 2.500000000000000000, -4.230127018922201998 ) ) ;
#86869=ORIENTED_EDGE ( 'NONE', *, *, #11996, .T. ) ;
#86870=FACE_OUTER_BOUND ( 'NONE', #85541, .T. ) ;
#86871=CIRCLE ( 'NONE', #120339, 2.000000000000000000 ) ;
#86872=CIRCLE ( 'NONE', #99422, 0.06509327318403745899 ) ;
#86873=DIRECTION ( 'NONE',  ( -0.000000000000000000, 1.000000000000000000, -0.000000000000000000 ) ) ;
#86874=CARTESIAN_POINT ( 'NONE',  ( -11.89999999999999503, 12.50000000000000000, 3.983716857408420076 ) ) ;
#86877=ORIENTED_EDGE ( 'NONE', *, *, #117610, .T. ) ;
#86878=AXIS2_PLACEMENT_3D ( 'NONE', #24389, #64304, #84596 ) ;
#86879=EDGE_CURVE ( 'NONE', #94866, #21053, #92167, .T. ) ;
#86880=ORIENTED_EDGE ( 'NONE', *, *, #34956, .F. ) ;
#86881=ORIENTED_EDGE ( 'NONE', *, *, #61884, .F. ) ;
#86882=ORIENTED_EDGE ( 'NONE', *, *, #99351, .T. ) ;
#86883=FACE_OUTER_BOUND ( 'NONE', #82279, .T. ) ;
#86884=AXIS2_PLACEMENT_3D ( 'NONE', #79498, #923, #110862 ) ;
#86885=DIRECTION ( 'NONE',  ( -0.05223670945016245515, 0.9986347311133432214, 0.000000000000000000 ) ) ;
#86886=CARTESIAN_POINT ( 'NONE',  ( -11.64999999999999680, 2.500000000000000000, -6.395190528383298378 ) ) ;
#86887=CIRCLE ( 'NONE', #128781, 0.1000000000000000056 ) ;
#86888=DIRECTION ( 'NONE',  ( 0.000000000000000000, 1.000000000000000000, 0.000000000000000000 ) ) ;
#86889=AXIS2_PLACEMENT_3D ( 'NONE', #10622, #79406, #108196 ) ;
#86890=VERTEX_POINT ( 'NONE', #2489 ) ;
#86891=CIRCLE ( 'NONE', #30493, 0.06509327318403745899 ) ;
#86892=CARTESIAN_POINT ( 'NONE',  ( 11.64999999999990266, 12.50000000000000000, -6.495190528383302464 ) ) ;
#86893=VECTOR ( 'NONE', #123713, 1000.000000000000000 ) ;
#86894=EDGE_LOOP ( 'NONE', ( #56976, #23396 ) ) ;
#86895=CARTESIAN_POINT ( 'NONE',  ( 5.849999999999933920, 2.500000000000000000, 5.802370205355744659 ) ) ;
#86896=DIRECTION ( 'NONE',  ( -0.000000000000000000, 1.000000000000000000, -0.000000000000000000 ) ) ;
#86897=LINE ( 'NONE', #86241, #455 ) ;
#86898=DIRECTION ( 'NONE',  ( 0.000000000000000000, 0.000000000000000000, 1.000000000000000000 ) ) ;
#86899=ADVANCED_FACE ( 'NONE', ( #101364 ), #66850, .T. ) ;
#86900=ORIENTED_EDGE ( 'NONE', *, *, #60821, .F. ) ;
#86902=EDGE_LOOP ( 'NONE', ( #24147, #51688 ) ) ;
#86903=ORIENTED_EDGE ( 'NONE', *, *, #60048, .T. ) ;
#86904=CARTESIAN_POINT ( 'NONE',  ( -4.800000000000024691, 12.50000000000000000, 4.676537180435972552 ) ) ;
#86905=CARTESIAN_POINT ( 'NONE',  ( 21.24754738303277435, 0.7337760880902381988, 4.182111650399361835 ) ) ;
#86906=EDGE_CURVE ( 'NONE', #89946, #83439, #68906, .T. ) ;
#86907=CARTESIAN_POINT ( 'NONE',  ( -6.450000000000017941, 2.500000000000000000, -2.611473670974877592 ) ) ;
#86908=FACE_BOUND ( 'NONE', #2068, .T. ) ;
#86909=DIRECTION ( 'NONE',  ( 0.000000000000000000, 0.000000000000000000, 1.000000000000000000 ) ) ;
#86910=DIRECTION ( 'NONE',  ( 0.000000000000000000, 0.000000000000000000, 1.000000000000000000 ) ) ;
#86911=DIRECTION ( 'NONE',  ( 0.000000000000000000, 0.000000000000000000, 1.000000000000000000 ) ) ;
#86912=CARTESIAN_POINT ( 'NONE',  ( -11.89999999999999503, 2.500000000000000000, 3.883716857408420431 ) ) ;
#86915=CARTESIAN_POINT ( 'NONE',  ( 1.899999999999951283, 2.500000000000000000, -0.3464101615137782364 ) ) ;
#86916=DIRECTION ( 'NONE',  ( -0.000000000000000000, -1.000000000000000000, -0.000000000000000000 ) ) ;
#86917=CONICAL_SURFACE ( 'NONE', #74411, 0.09999999999999982514, 0.003490658503988666988 ) ;
#86918=VECTOR ( 'NONE', #11431, 1000.000000000000000 ) ;
#86919=FACE_OUTER_BOUND ( 'NONE', #51932, .T. ) ;
#86920=AXIS2_PLACEMENT_3D ( 'NONE', #88357, #47175, #65509 ) ;
#86921=ADVANCED_FACE ( 'NONE', ( #81078 ), #62732, .T. ) ;
#86922=ORIENTED_EDGE ( 'NONE', *, *, #115253, .T. ) ;
#86923=ORIENTED_EDGE ( 'NONE', *, *, #69895, .F. ) ;
#86924=ORIENTED_EDGE ( 'NONE', *, *, #104781, .T. ) ;
#86925=ORIENTED_EDGE ( 'NONE', *, *, #111527, .T. ) ;
#86926=DIRECTION ( 'NONE',  ( 0.000000000000000000, 0.000000000000000000, 1.000000000000000000 ) ) ;
#86927=FACE_BOUND ( 'NONE', #93350, .T. ) ;
#86928=FACE_OUTER_BOUND ( 'NONE', #38310, .T. ) ;
#86929=CIRCLE ( 'NONE', #24158, 0.1000000000000000472 ) ;
#86930=CARTESIAN_POINT ( 'NONE',  ( 11.69999999999990870, 2.500000000000000000, -4.430127018922202176 ) ) ;
#86931=EDGE_CURVE ( 'NONE', #120557, #46758, #14246, .T. ) ;
#86932=AXIS2_PLACEMENT_3D ( 'NONE', #45784, #67305, #17584 ) ;
#86933=CIRCLE ( 'NONE', #30533, 0.1000000000000002554 ) ;
#86934=ORIENTED_EDGE ( 'NONE', *, *, #52894, .F. ) ;
#86935=EDGE_CURVE ( 'NONE', #64023, #781, #112838, .T. ) ;
#86936=CARTESIAN_POINT ( 'NONE',  ( 10.59999999999991260, 2.500000000000000000, -0.3464101615137783474 ) ) ;
#86937=ADVANCED_FACE ( 'NONE', ( #125497 ), #84284, .T. ) ;
#86938=DIRECTION ( 'NONE',  ( -4.274815082592931898E-19, -0.9999939076577903929, -0.003490651415223739937 ) ) ;
#86939=EDGE_CURVE ( 'NONE', #74400, #27754, #87686, .T. ) ;
#86940=EDGE_CURVE ( 'NONE', #594, #55743, #119094, .T. ) ;
#86941=VERTEX_POINT ( 'NONE', #105864 ) ;
#86942=CARTESIAN_POINT ( 'NONE',  ( 1.449999999999952216, 12.50000000000000000, 1.818653347947321475 ) ) ;
#86943=CARTESIAN_POINT ( 'NONE',  ( 20.59313469514036399, 2.666874593322338338, -2.243770147468779896 ) ) ;
#86944=CIRCLE ( 'NONE', #92939, 0.09999999999999982514 ) ;
#86945=AXIS2_PLACEMENT_3D ( 'NONE', #96285, #125738, #73428 ) ;
#86946=ADVANCED_FACE ( 'NONE', ( #16167 ), #37533, .T. ) ;
#86947=EDGE_LOOP ( 'NONE', ( #63803, #63771, #83846, #123647 ) ) ;
#86948=DIRECTION ( 'NONE',  ( -0.000000000000000000, 1.000000000000000000, -0.000000000000000000 ) ) ;
#86950=CARTESIAN_POINT ( 'NONE',  ( 6.249999999999932498, 2.500000000000000000, -2.857883832488653741 ) ) ;
#86951=EDGE_CURVE ( 'NONE', #64286, #113932, #54817, .T. ) ;
#86952=VERTEX_POINT ( 'NONE', #124218 ) ;
#86953=DIRECTION ( 'NONE',  ( 0.000000000000000000, 0.000000000000000000, 1.000000000000000000 ) ) ;
#86955=FACE_OUTER_BOUND ( 'NONE', #98322, .T. ) ;
#86956=ORIENTED_EDGE ( 'NONE', *, *, #75664, .T. ) ;
#86957=CARTESIAN_POINT ( 'NONE',  ( 13.14999999999990088, 12.50000000000000000, 2.576566944158910744 ) ) ;
#86958=ORIENTED_EDGE ( 'NONE', *, *, #13919, .F. ) ;
#86959=ORIENTED_EDGE ( 'NONE', *, *, #128714, .T. ) ;
#86960=DIRECTION ( 'NONE',  ( -0.000000000000000000, 1.000000000000000000, -0.000000000000000000 ) ) ;
#86961=EDGE_CURVE ( 'NONE', #102321, #125657, #25004, .T. ) ;
#86962=ORIENTED_EDGE ( 'NONE', *, *, #25058, .F. ) ;
#86963=DIRECTION ( 'NONE',  ( 0.000000000000000000, 1.000000000000000000, 0.000000000000000000 ) ) ;
#86964=DIRECTION ( 'NONE',  ( 0.000000000000000000, 0.000000000000000000, -1.000000000000000000 ) ) ;
#86965=AXIS2_PLACEMENT_3D ( 'NONE', #95030, #54441, #93738 ) ;
#86966=ORIENTED_EDGE ( 'NONE', *, *, #38854, .F. ) ;
#86967=CIRCLE ( 'NONE', #76514, 0.06509327318403741736 ) ;
#86968=DIRECTION ( 'NONE',  ( 0.000000000000000000, 1.000000000000000000, 0.000000000000000000 ) ) ;
#86969=VERTEX_POINT ( 'NONE', #44359 ) ;
#86970=CARTESIAN_POINT ( 'NONE',  ( 7.499999999999925393, 2.500000000000000000, 4.922947341949748257 ) ) ;
#86971=DIRECTION ( 'NONE',  ( 0.000000000000000000, 0.000000000000000000, 1.000000000000000000 ) ) ;
#86972=DIRECTION ( 'NONE',  ( 0.000000000000000000, 0.000000000000000000, 1.000000000000000000 ) ) ;
#86973=DIRECTION ( 'NONE',  ( 0.000000000000000000, 0.000000000000000000, 1.000000000000000000 ) ) ;
#86974=CARTESIAN_POINT ( 'NONE',  ( 12.49999999999990585, 12.50000000000000000, 3.572213422710607489 ) ) ;
#86975=CIRCLE ( 'NONE', #103720, 0.06509327318403745899 ) ;
#86976=ORIENTED_EDGE ( 'NONE', *, *, #102788, .F. ) ;
#86977=ORIENTED_EDGE ( 'NONE', *, *, #44102, .F. ) ;
#86978=CARTESIAN_POINT ( 'NONE',  ( -9.600000000000006750, 2.500000000000000000, -0.6928203230275542523 ) ) ;
#86979=CARTESIAN_POINT ( 'NONE',  ( 0.6499999999999566125, 2.500000000000000000, -6.248780366869526759 ) ) ;
#86980=CARTESIAN_POINT ( 'NONE',  ( -9.600000000000006750, 2.500000000000000000, 0.6928203230275494784 ) ) ;
#86981=ORIENTED_EDGE ( 'NONE', *, *, #9692, .T. ) ;
#86982=ORIENTED_EDGE ( 'NONE', *, *, #88908, .F. ) ;
#86983=VERTEX_POINT ( 'NONE', #53550 ) ;
#86984=DIRECTION ( 'NONE',  ( 0.000000000000000000, 0.000000000000000000, 1.000000000000000000 ) ) ;
#86985=VECTOR ( 'NONE', #96350, 1000.000000000000000 ) ;
#86986=DIRECTION ( 'NONE',  ( 0.000000000000000000, 0.000000000000000000, 1.000000000000000000 ) ) ;
#86987=CARTESIAN_POINT ( 'NONE',  ( -1.250000000000001554, 2.500000000000000000, 6.495190528383297135 ) ) ;
#86988=AXIS2_PLACEMENT_3D ( 'NONE', #5992, #7932, #47239 ) ;
#86990=CARTESIAN_POINT ( 'NONE',  ( -5.850000000000018296, 2.500000000000000000, 1.372243186433545370 ) ) ;
#86991=CARTESIAN_POINT ( 'NONE',  ( -6.900000000000015454, 12.50000000000000000, 3.983716857408420076 ) ) ;
#86992=DIRECTION ( 'NONE',  ( 0.000000000000000000, 0.000000000000000000, 1.000000000000000000 ) ) ;
#86993=DIRECTION ( 'NONE',  ( -0.000000000000000000, -1.000000000000000000, -0.000000000000000000 ) ) ;
#86994=FACE_OUTER_BOUND ( 'NONE', #90802, .T. ) ;
#86995=CARTESIAN_POINT ( 'NONE',  ( -5.850000000000021849, 2.500000000000000000, -1.472243186433550122 ) ) ;
#86996=VERTEX_POINT ( 'NONE', #65280 ) ;
#86997=EDGE_CURVE ( 'NONE', #124869, #32548, #56387, .T. ) ;
#86998=ADVANCED_FACE ( 'NONE', ( #43748 ), #47997, .T. ) ;
#86999=CARTESIAN_POINT ( 'NONE',  ( 6.699999999999930012, 2.500000000000000000, -4.230127018922201998 ) ) ;
#87001=ORIENTED_EDGE ( 'NONE', *, *, #39372, .T. ) ;
#87002=DIRECTION ( 'NONE',  ( 0.000000000000000000, -0.000000000000000000, 1.000000000000000000 ) ) ;
#87003=DIRECTION ( 'NONE',  ( 0.000000000000000000, 0.000000000000000000, -1.000000000000000000 ) ) ;
#87004=CONICAL_SURFACE ( 'NONE', #74490, 0.1000000000000002554, 0.003490658503988666988 ) ;
#87005=LINE ( 'NONE', #37281, #105111 ) ;
#87006=DIRECTION ( 'NONE',  ( 0.000000000000000000, -0.9999939076577903929, 0.003490651415223739937 ) ) ;
#87008=DIRECTION ( 'NONE',  ( 0.000000000000000000, 0.000000000000000000, 1.000000000000000000 ) ) ;
#87009=DIRECTION ( 'NONE',  ( 0.000000000000000000, 1.000000000000000000, 0.000000000000000000 ) ) ;
#87010=AXIS2_PLACEMENT_3D ( 'NONE', #105693, #56567, #96485 ) ;
#87011=DIRECTION ( 'NONE',  ( 0.000000000000000000, 1.000000000000000000, 0.000000000000000000 ) ) ;
#87012=EDGE_LOOP ( 'NONE', ( #96296, #30262 ) ) ;
#87013=CARTESIAN_POINT ( 'NONE',  ( 9.399999999999918643, 2.500000000000000000, 0.2464101615137736789 ) ) ;
#87014=AXIS2_PLACEMENT_3D ( 'NONE', #114485, #45117, #35301 ) ;
#87015=AXIS2_PLACEMENT_3D ( 'NONE', #9673, #11602, #31899 ) ;
#87016=CIRCLE ( 'NONE', #128908, 0.09999999999999982514 ) ;
#87017=CARTESIAN_POINT ( 'NONE',  ( -11.44999999999999751, 12.50000000000000000, -2.511473670974873951 ) ) ;
#87018=ORIENTED_EDGE ( 'NONE', *, *, #29432, .F. ) ;
#87020=VERTEX_POINT ( 'NONE', #123552 ) ;
#87021=VERTEX_POINT ( 'NONE', #85575 ) ;
#87022=ORIENTED_EDGE ( 'NONE', *, *, #123175, .F. ) ;
#87023=CARTESIAN_POINT ( 'NONE',  ( -4.293440603042597559E-14, 2.500000000000000000, 5.122947341949749323 ) ) ;
#87024=CARTESIAN_POINT ( 'NONE',  ( -5.600000000000020073, 2.500000000000000000, -0.3464101615137782364 ) ) ;
#87025=CONICAL_SURFACE ( 'NONE', #24341, 0.1000000000000002554, 0.003490658503988666988 ) ;
#87026=ORIENTED_EDGE ( 'NONE', *, *, #37970, .T. ) ;
#87027=DIRECTION ( 'NONE',  ( 0.000000000000000000, 0.000000000000000000, -1.000000000000000000 ) ) ;
#87028=LINE ( 'NONE', #106667, #8950 ) ;
#87029=CIRCLE ( 'NONE', #45280, 0.09999999999999982514 ) ;
#87030=CONICAL_SURFACE ( 'NONE', #122551, 0.1000000000000002554, 0.003490658503988666988 ) ;
#87031=CARTESIAN_POINT ( 'NONE',  ( 0.5999999999999612310, 2.500000000000000000, -0.3464101615137760715 ) ) ;
#87032=ORIENTED_EDGE ( 'NONE', *, *, #115766, .F. ) ;
#87033=LINE ( 'NONE', #88307, #5566 ) ;
#87034=CARTESIAN_POINT ( 'NONE',  ( 1.049999999999952971, 2.500000000000000000, 6.048780366869521252 ) ) ;
#87035=EDGE_CURVE ( 'NONE', #120902, #515, #79389, .T. ) ;
#87036=ORIENTED_EDGE ( 'NONE', *, *, #24549, .T. ) ;
#87037=VERTEX_POINT ( 'NONE', #113761 ) ;
#87038=ORIENTED_EDGE ( 'NONE', *, *, #95360, .F. ) ;
#87039=FACE_OUTER_BOUND ( 'NONE', #26640, .T. ) ;
#87040=PLANE ( 'NONE',  #46053 ) ;
#87041=ADVANCED_FACE ( 'NONE', ( #114383 ), #4066, .T. ) ;
#87042=EDGE_LOOP ( 'NONE', ( #114745, #63065 ) ) ;
#87043=DIRECTION ( 'NONE',  ( -0.000000000000000000, -1.000000000000000000, -0.000000000000000000 ) ) ;
#87044=FACE_OUTER_BOUND ( 'NONE', #31910, .T. ) ;
#87045=CARTESIAN_POINT ( 'NONE',  ( 5.399999999999932854, 2.500000000000000000, 3.637306695894644726 ) ) ;
#87046=CARTESIAN_POINT ( 'NONE',  ( 11.04999999999990834, 12.50000000000000000, 1.753560074763284016 ) ) ;
#87047=ADVANCED_FACE ( 'NONE', ( #45023 ), #43803, .T. ) ;
#87048=ORIENTED_EDGE ( 'NONE', *, *, #6333, .F. ) ;
#87049=CIRCLE ( 'NONE', #72499, 0.06509327318403745899 ) ;
#87050=DIRECTION ( 'NONE',  ( 0.000000000000000000, 0.000000000000000000, 1.000000000000000000 ) ) ;
#87051=CIRCLE ( 'NONE', #20164, 0.06509327318403745899 ) ;
#87052=ORIENTED_EDGE ( 'NONE', *, *, #79697, .F. ) ;
#87053=EDGE_LOOP ( 'NONE', ( #6497, #23342, #10353, #89310 ) ) ;
#87054=ORIENTED_EDGE ( 'NONE', *, *, #303, .F. ) ;
#87055=EDGE_CURVE ( 'NONE', #113182, #111375, #116924, .T. ) ;
#87056=FACE_OUTER_BOUND ( 'NONE', #76118, .T. ) ;
#87057=FACE_BOUND ( 'NONE', #121916, .T. ) ;
#87058=CARTESIAN_POINT ( 'NONE',  ( 8.099999999999921485, 2.500000000000000000, -0.3464101615137783474 ) ) ;
#87059=CARTESIAN_POINT ( 'NONE',  ( -8.350000000000013856, 2.500000000000000000, -6.595190528383296780 ) ) ;
#87060=AXIS2_PLACEMENT_3D ( 'NONE', #50499, #59047, #90412 ) ;
#87061=CONICAL_SURFACE ( 'NONE', #91276, 0.09999999999999982514, 0.003490658503988666988 ) ;
#87062=DIRECTION ( 'NONE',  ( 0.000000000000000000, 0.000000000000000000, -1.000000000000000000 ) ) ;
#87063=ORIENTED_EDGE ( 'NONE', *, *, #102019, .F. ) ;
#87064=LINE ( 'NONE', #127011, #361 ) ;
#87065=CARTESIAN_POINT ( 'NONE',  ( -12.89999999999999325, 2.500000000000000000, -3.637306695894647390 ) ) ;
#87066=CARTESIAN_POINT ( 'NONE',  ( 1.449999999999951772, 2.500000000000000000, -6.148780366869526226 ) ) ;
#87067=DIRECTION ( 'NONE',  ( 0.000000000000000000, 0.000000000000000000, 1.000000000000000000 ) ) ;
#87068=VERTEX_POINT ( 'NONE', #27945 ) ;
#87069=CIRCLE ( 'NONE', #124834, 0.1000000000000002554 ) ;
#87070=DIRECTION ( 'NONE',  ( -4.274815082592931898E-19, -0.9999939076577903929, -0.003490651415223739937 ) ) ;
#87071=AXIS2_PLACEMENT_3D ( 'NONE', #32769, #41930, #73298 ) ;
#87073=EDGE_LOOP ( 'NONE', ( #41059, #36482 ) ) ;
#87074=CARTESIAN_POINT ( 'NONE',  ( 3.949999999999940670, 2.500000000000000000, 1.918653347947321564 ) ) ;
#87075=LINE ( 'NONE', #77899, #69393 ) ;
#87076=FACE_BOUND ( 'NONE', #10637, .T. ) ;
#87077=CARTESIAN_POINT ( 'NONE',  ( -10.65000000000000391, 2.500000000000000000, -6.841600689897075149 ) ) ;
#87078=EDGE_CURVE ( 'NONE', #118132, #112463, #6992, .T. ) ;
#87079=ORIENTED_EDGE ( 'NONE', *, *, #93483, .F. ) ;
#87080=CARTESIAN_POINT ( 'NONE',  ( -4.150000000000025224, 2.500000000000000000, 5.902370205355745192 ) ) ;
#87081=EDGE_LOOP ( 'NONE', ( #96578, #102388 ) ) ;
#87082=EDGE_LOOP ( 'NONE', ( #25473, #17811, #108064, #114366 ) ) ;
#87083=CARTESIAN_POINT ( 'NONE',  ( 16.55874544816229488, 0.4845305829427787869, -6.091953208798931207 ) ) ;
#87084=ADVANCED_FACE ( 'NONE', ( #97331 ), #16660, .T. ) ;
#87086=VECTOR ( 'NONE', #124152, 1000.000000000000000 ) ;
#87087=ADVANCED_FACE ( 'NONE', ( #128088 ), #86202, .T. ) ;
#87088=ORIENTED_EDGE ( 'NONE', *, *, #8614, .T. ) ;
#87089=CARTESIAN_POINT ( 'NONE',  ( -5.850000000000021849, 2.500000000000000000, -7.188010851410854052 ) ) ;
#87090=AXIS2_PLACEMENT_3D ( 'NONE', #94518, #15945, #104969 ) ;
#87091=CARTESIAN_POINT ( 'NONE',  ( -10.84999999999999964, 2.500000000000000000, 1.372243186433545370 ) ) ;
#87092=CONICAL_SURFACE ( 'NONE', #116335, 0.1000000000000002554, 0.003490658503988666988 ) ;
#87093=EDGE_CURVE ( 'NONE', #76525, #79082, #7646, .T. ) ;
#87094=ADVANCED_FACE ( 'NONE', ( #47599 ), #86859, .T. ) ;
#87095=DIRECTION ( 'NONE',  ( 0.000000000000000000, -0.000000000000000000, 1.000000000000000000 ) ) ;
#87096=ADVANCED_FACE ( 'NONE', ( #77050 ), #6200, .T. ) ;
#87097=CONICAL_SURFACE ( 'NONE', #62087, 0.09999999999999982514, 0.003490658503988666988 ) ;
#87098=VECTOR ( 'NONE', #104790, 1000.000000000000000 ) ;
#87099=ORIENTED_EDGE ( 'NONE', *, *, #39111, .F. ) ;
#87100=CIRCLE ( 'NONE', #30706, 0.1000000000000000472 ) ;
#87101=DIRECTION ( 'NONE',  ( 0.000000000000000000, -0.000000000000000000, 1.000000000000000000 ) ) ;
#87102=ADVANCED_FACE ( 'NONE', ( #68508 ), #58468, .T. ) ;
#87103=CARTESIAN_POINT ( 'NONE',  ( -11.05000000000000071, 2.500000000000000000, -6.941600689897075682 ) ) ;
#87104=CARTESIAN_POINT ( 'NONE',  ( -5.800000000000018474, 12.50000000000000000, 0.06509327318403515528 ) ) ;
#87105=CARTESIAN_POINT ( 'NONE',  ( 3.349999999999941913, 2.500000000000000000, 6.495190528383297135 ) ) ;
#87106=VERTEX_POINT ( 'NONE', #96666 ) ;
#87107=DIRECTION ( 'NONE',  ( 0.000000000000000000, 0.000000000000000000, -1.000000000000000000 ) ) ;
#87108=EDGE_LOOP ( 'NONE', ( #9299, #125558, #16192, #1346 ) ) ;
#87109=AXIS2_PLACEMENT_3D ( 'NONE', #51733, #41278, #81192 ) ;
#87110=CARTESIAN_POINT ( 'NONE',  ( 7.949999999999925571, 12.50000000000000000, -6.560283801567339701 ) ) ;
#87111=DIRECTION ( 'NONE',  ( 0.000000000000000000, 0.000000000000000000, 1.000000000000000000 ) ) ;
#87112=EDGE_CURVE ( 'NONE', #121932, #54992, #118256, .T. ) ;
#87113=CIRCLE ( 'NONE', #97578, 0.06509327318403745899 ) ;
#87114=ORIENTED_EDGE ( 'NONE', *, *, #118281, .T. ) ;
#87115=DIRECTION ( 'NONE',  ( 0.000000000000000000, 0.000000000000000000, 1.000000000000000000 ) ) ;
#87116=DIRECTION ( 'NONE',  ( -0.000000000000000000, -1.000000000000000000, -0.000000000000000000 ) ) ;
#87117=DIRECTION ( 'NONE',  ( 0.000000000000000000, 1.000000000000000000, 0.000000000000000000 ) ) ;
#87118=VECTOR ( 'NONE', #95500, 1000.000000000000000 ) ;
#87119=LINE ( 'NONE', #46544, #119733 ) ;
#87120=ORIENTED_EDGE ( 'NONE', *, *, #106115, .F. ) ;
#87121=DIRECTION ( 'NONE',  ( -0.000000000000000000, 1.000000000000000000, -0.000000000000000000 ) ) ;
#87122=DIRECTION ( 'NONE',  ( 0.000000000000000000, 0.000000000000000000, 1.000000000000000000 ) ) ;
#87123=DIRECTION ( 'NONE',  ( 0.000000000000000000, -0.000000000000000000, 1.000000000000000000 ) ) ;
#87124=CARTESIAN_POINT ( 'NONE',  ( 7.099999999999928590, 2.500000000000000000, -4.430127018922202176 ) ) ;
#87125=DIRECTION ( 'NONE',  ( 0.000000000000000000, 0.000000000000000000, 1.000000000000000000 ) ) ;
#87126=EDGE_LOOP ( 'NONE', ( #58130, #61020 ) ) ;
#87127=ORIENTED_EDGE ( 'NONE', *, *, #100776, .F. ) ;
#87128=LINE ( 'NONE', #55740, #9435 ) ;
#87129=ORIENTED_EDGE ( 'NONE', *, *, #68620, .F. ) ;
#87130=FACE_OUTER_BOUND ( 'NONE', #19963, .T. ) ;
#87131=EDGE_LOOP ( 'NONE', ( #48096, #49625, #27265, #50150 ) ) ;
#87132=EDGE_LOOP ( 'NONE', ( #105689, #89667 ) ) ;
#87133=VERTEX_POINT ( 'NONE', #116308 ) ;
#87134=VECTOR ( 'NONE', #94690, 1000.000000000000000 ) ;
#87135=DIRECTION ( 'NONE',  ( -0.000000000000000000, -1.000000000000000000, -0.000000000000000000 ) ) ;
#87136=FACE_OUTER_BOUND ( 'NONE', #34823, .T. ) ;
#87137=DIRECTION ( 'NONE',  ( -0.000000000000000000, 1.000000000000000000, -0.000000000000000000 ) ) ;
#87138=CARTESIAN_POINT ( 'NONE',  ( -1.250000000000035749, 12.50000000000000000, -2.857883832488653741 ) ) ;
#87139=CARTESIAN_POINT ( 'NONE',  ( -2.100000000000034728, 2.500000000000000000, 4.430127018922196847 ) ) ;
#87140=CARTESIAN_POINT ( 'NONE',  ( -14.19999999999998685, 2.500000000000000000, 0.09999999999999989453 ) ) ;
#87141=EDGE_LOOP ( 'NONE', ( #3350, #45635 ) ) ;
#87142=CARTESIAN_POINT ( 'NONE',  ( -4.150000000000024336, 12.50000000000000000, -2.922977105672691422 ) ) ;
#87143=VERTEX_POINT ( 'NONE', #46958 ) ;
#87144=AXIS2_PLACEMENT_3D ( 'NONE', #47710, #78471, #118364 ) ;
#87145=ORIENTED_EDGE ( 'NONE', *, *, #52833, .F. ) ;
#87146=ORIENTED_EDGE ( 'NONE', *, *, #34177, .T. ) ;
#87147=ADVANCED_FACE ( 'NONE', ( #108430 ), #35481, .T. ) ;
#87148=VERTEX_POINT ( 'NONE', #8934 ) ;
#87149=AXIS2_PLACEMENT_3D ( 'NONE', #117436, #3180, #76904 ) ;
#87150=DIRECTION ( 'NONE',  ( 0.000000000000000000, 0.000000000000000000, 1.000000000000000000 ) ) ;
#87151=ORIENTED_EDGE ( 'NONE', *, *, #109463, .T. ) ;
#87152=ORIENTED_EDGE ( 'NONE', *, *, #59197, .T. ) ;
#87153=AXIS2_PLACEMENT_3D ( 'NONE', #111162, #12962, #82391 ) ;
#87154=EDGE_CURVE ( 'NONE', #110307, #93392, #100314, .T. ) ;
#87155=CARTESIAN_POINT ( 'NONE',  ( 11.84999999999990727, 12.50000000000000000, -1.883746621131363597 ) ) ;
#87156=LINE ( 'NONE', #127731, #123163 ) ;
#87157=CARTESIAN_POINT ( 'NONE',  ( 0.8499999999999557909, 2.500000000000000000, -6.595190528383302109 ) ) ;
#87158=DIRECTION ( 'NONE',  ( -4.274815082592931898E-19, -0.9999939076577903929, -0.003490651415223739937 ) ) ;
#87159=DIRECTION ( 'NONE',  ( 0.000000000000000000, 1.000000000000000000, 0.000000000000000000 ) ) ;
#87160=VERTEX_POINT ( 'NONE', #57413 ) ;
#87161=DIRECTION ( 'NONE',  ( 0.000000000000000000, 1.000000000000000000, 0.000000000000000000 ) ) ;
#87162=AXIS2_PLACEMENT_3D ( 'NONE', #97976, #28609, #128760 ) ;
#87163=ORIENTED_EDGE ( 'NONE', *, *, #128667, .T. ) ;
#87164=DIRECTION ( 'NONE',  ( 0.000000000000000000, 0.000000000000000000, 1.000000000000000000 ) ) ;
#87165=CIRCLE ( 'NONE', #126890, 0.1000000000000002554 ) ;
#87167=FACE_OUTER_BOUND ( 'NONE', #53463, .T. ) ;
#87168=ORIENTED_EDGE ( 'NONE', *, *, #103485, .T. ) ;
#87169=VERTEX_POINT ( 'NONE', #6339 ) ;
#87170=CARTESIAN_POINT ( 'NONE',  ( 6.849999999999929479, 12.50000000000000000, -1.753560074763288679 ) ) ;
#87171=DIRECTION ( 'NONE',  ( -4.274815082592931898E-19, -0.9999939076577903929, -0.003490651415223739937 ) ) ;
#87172=DIRECTION ( 'NONE',  ( 0.000000000000000000, 0.000000000000000000, 1.000000000000000000 ) ) ;
#87173=DIRECTION ( 'NONE',  ( 0.000000000000000000, 0.000000000000000000, 1.000000000000000000 ) ) ;
#87174=DIRECTION ( 'NONE',  ( -4.274815082592931898E-19, -0.9999939076577903929, -0.003490651415223739937 ) ) ;
#87175=ORIENTED_EDGE ( 'NONE', *, *, #93804, .F. ) ;
#87176=CARTESIAN_POINT ( 'NONE',  ( 11.89999999999990443, 2.500000000000000000, 0.3464101615137736845 ) ) ;
#87177=CARTESIAN_POINT ( 'NONE',  ( -10.60000000000000142, 2.500000000000000000, -0.3464101615137782364 ) ) ;
#87178=DIRECTION ( 'NONE',  ( 0.000000000000000000, 0.000000000000000000, -1.000000000000000000 ) ) ;
#87179=CARTESIAN_POINT ( 'NONE',  ( 13.94999999999989626, 2.500000000000000000, 2.511473670974873507 ) ) ;
#87181=CONICAL_SURFACE ( 'NONE', #70468, 0.09999999999999999167, 0.003490658503988666988 ) ;
#87182=CARTESIAN_POINT ( 'NONE',  ( -2.700000000000029932, 12.50000000000000000, -4.676537180435977881 ) ) ;
#87183=EDGE_CURVE ( 'NONE', #45516, #87698, #91905, .T. ) ;
#87184=ORIENTED_EDGE ( 'NONE', *, *, #114862, .T. ) ;
#87185=CIRCLE ( 'NONE', #78813, 0.1000000000000002554 ) ;
#87186=ORIENTED_EDGE ( 'NONE', *, *, #62556, .T. ) ;
#87187=CARTESIAN_POINT ( 'NONE',  ( 3.099999999999944134, 12.50000000000000000, 4.676537180435972552 ) ) ;
#87188=CIRCLE ( 'NONE', #103934, 0.1000000000000002554 ) ;
#87189=EDGE_LOOP ( 'NONE', ( #56148, #107283, #102596, #109446 ) ) ;
#87190=CIRCLE ( 'NONE', #7775, 0.06509327318403745899 ) ;
#87191=CARTESIAN_POINT ( 'NONE',  ( -8.750000000000005329, 2.500000000000000000, 5.902370205355745192 ) ) ;
#87192=CARTESIAN_POINT ( 'NONE',  ( -4.600000000000024514, 12.50000000000000000, 3.702399969078682407 ) ) ;
#87193=ADVANCED_FACE ( 'NONE', ( #48233 ), #102376, .T. ) ;
#87194=CIRCLE ( 'NONE', #16170, 0.1000000000000000056 ) ;
#87195=ADVANCED_FACE ( 'NONE', ( #124640 ), #89930, .T. ) ;
#87196=ORIENTED_EDGE ( 'NONE', *, *, #19233, .F. ) ;
#87198=DIRECTION ( 'NONE',  ( 0.000000000000000000, 0.000000000000000000, 1.000000000000000000 ) ) ;
#87199=AXIS2_PLACEMENT_3D ( 'NONE', #7766, #37881, #117703 ) ;
#87200=DIRECTION ( 'NONE',  ( 0.000000000000000000, -0.000000000000000000, 1.000000000000000000 ) ) ;
#87201=EDGE_CURVE ( 'NONE', #47551, #25742, #73220, .T. ) ;
#87202=DIRECTION ( 'NONE',  ( 0.000000000000000000, 1.000000000000000000, 0.000000000000000000 ) ) ;
#87203=ORIENTED_EDGE ( 'NONE', *, *, #101293, .F. ) ;
#87204=AXIS2_PLACEMENT_3D ( 'NONE', #96474, #84742, #64451 ) ;
#87206=DIRECTION ( 'NONE',  ( -4.274815082592931898E-19, -0.9999939076577903929, -0.003490651415223739937 ) ) ;
#87207=PLANE ( 'NONE',  #125030 ) ;
#87208=ADVANCED_FACE ( 'NONE', ( #33680 ), #66350, .T. ) ;
#87209=ORIENTED_EDGE ( 'NONE', *, *, #33082, .T. ) ;
#87210=EDGE_CURVE ( 'NONE', #64313, #37202, #87774, .T. ) ;
#87213=FACE_OUTER_BOUND ( 'NONE', #13331, .T. ) ;
#87214=ORIENTED_EDGE ( 'NONE', *, *, #121501, .F. ) ;
#87215=CARTESIAN_POINT ( 'NONE',  ( 4.599999999999936584, 2.500000000000000000, 4.330127018922196314 ) ) ;
#87216=VERTEX_POINT ( 'NONE', #84707 ) ;
#87217=CARTESIAN_POINT ( 'NONE',  ( 13.74999999999993427, 12.50000000000000000, 2.230156782645134950 ) ) ;
#87218=CARTESIAN_POINT ( 'NONE',  ( 4.999999999999971578, 12.50000000000000000, 0.06509327318403515528 ) ) ;
#87219=CIRCLE ( 'NONE', #108152, 0.1000000000000002554 ) ;
#87220=FACE_OUTER_BOUND ( 'NONE', #25414, .T. ) ;
#87221=VERTEX_POINT ( 'NONE', #16595 ) ;
#87222=DIRECTION ( 'NONE',  ( 0.000000000000000000, 1.000000000000000000, 0.000000000000000000 ) ) ;
#87223=DIRECTION ( 'NONE',  ( 0.000000000000000000, 0.000000000000000000, -1.000000000000000000 ) ) ;
#87224=EDGE_LOOP ( 'NONE', ( #89890, #96845, #120056, #59454 ) ) ;
#87225=DIRECTION ( 'NONE',  ( 0.000000000000000000, -0.000000000000000000, 1.000000000000000000 ) ) ;
#87226=ORIENTED_EDGE ( 'NONE', *, *, #13062, .T. ) ;
#87227=DIRECTION ( 'NONE',  ( 0.000000000000000000, -0.000000000000000000, 1.000000000000000000 ) ) ;
#87228=ADVANCED_FACE ( 'NONE', ( #34991 ), #66931, .T. ) ;
#87229=VERTEX_POINT ( 'NONE', #96444 ) ;
#87230=CARTESIAN_POINT ( 'NONE',  ( 6.899999999999928413, 2.500000000000000000, 3.983716857408420964 ) ) ;
#87231=DIRECTION ( 'NONE',  ( 0.000000000000000000, 0.000000000000000000, 1.000000000000000000 ) ) ;
#87232=VERTEX_POINT ( 'NONE', #65709 ) ;
#87233=EDGE_LOOP ( 'NONE', ( #113571, #77392 ) ) ;
#87234=DIRECTION ( 'NONE',  ( -4.274815082592931898E-19, -0.9999939076577903929, -0.003490651415223739937 ) ) ;
#87235=DIRECTION ( 'NONE',  ( -0.000000000000000000, 1.000000000000000000, -0.000000000000000000 ) ) ;
#87236=ORIENTED_EDGE ( 'NONE', *, *, #22675, .F. ) ;
#87237=AXIS2_PLACEMENT_3D ( 'NONE', #51638, #73841, #121643 ) ;
#87238=EDGE_CURVE ( 'NONE', #82307, #98236, #6757, .T. ) ;
#87239=CARTESIAN_POINT ( 'NONE',  ( -2.100000000000033396, 2.500000000000000000, 0.5928203230275495006 ) ) ;
#87240=DIRECTION ( 'NONE',  ( 0.000000000000000000, -0.9999939076577903929, 0.003490651415223739937 ) ) ;
#87241=CONICAL_SURFACE ( 'NONE', #32989, 0.1000000000000002554, 0.003490658503988666988 ) ;
#87242=CARTESIAN_POINT ( 'NONE',  ( -3.950000000000028155, 2.500000000000000000, -6.941600689897077459 ) ) ;
#87243=DIRECTION ( 'NONE',  ( 0.000000000000000000, 1.000000000000000000, 0.000000000000000000 ) ) ;
#87244=EDGE_CURVE ( 'NONE', #35273, #37478, #44799, .T. ) ;
#87245=DIRECTION ( 'NONE',  ( 0.000000000000000000, 0.000000000000000000, -1.000000000000000000 ) ) ;
#87246=DIRECTION ( 'NONE',  ( 0.000000000000000000, -0.000000000000000000, 1.000000000000000000 ) ) ;
#87247=EDGE_CURVE ( 'NONE', #121877, #55444, #117008, .T. ) ;
#87248=AXIS2_PLACEMENT_3D ( 'NONE', #21198, #91878, #109591 ) ;
#87249=CIRCLE ( 'NONE', #66327, 0.06509327318403745899 ) ;
#87250=ADVANCED_FACE ( 'NONE', ( #14660 ), #114961, .T. ) ;
#87251=VERTEX_POINT ( 'NONE', #123347 ) ;
#87252=EDGE_LOOP ( 'NONE', ( #43568, #58213 ) ) ;
#87253=EDGE_CURVE ( 'NONE', #104830, #121148, #73585, .T. ) ;
#87254=ORIENTED_EDGE ( 'NONE', *, *, #66899, .T. ) ;
#87255=VERTEX_POINT ( 'NONE', #103717 ) ;
#87256=PLANE ( 'NONE',  #83078 ) ;
#87257=DIRECTION ( 'NONE',  ( 0.000000000000000000, 0.000000000000000000, 1.000000000000000000 ) ) ;
#87258=CARTESIAN_POINT ( 'NONE',  ( 13.74999999999989342, 12.50000000000000000, -1.537336459617587581 ) ) ;
#87259=ORIENTED_EDGE ( 'NONE', *, *, #5064, .T. ) ;
#87260=FACE_BOUND ( 'NONE', #5002, .T. ) ;
#87261=CARTESIAN_POINT ( 'NONE',  ( 9.399999999999918643, 12.50000000000000000, -0.3464101615137782364 ) ) ;
#87262=PLANE ( 'NONE',  #91877 ) ;
#87263=ADVANCED_FACE ( 'NONE', ( #76185 ), #75264, .T. ) ;
#87264=DIRECTION ( 'NONE',  ( 0.000000000000000000, 1.000000000000000000, 0.000000000000000000 ) ) ;
#87265=AXIS2_PLACEMENT_3D ( 'NONE', #15296, #34986, #114172 ) ;
#87266=EDGE_CURVE ( 'NONE', #27091, #50160, #23871, .T. ) ;
#87267=DIRECTION ( 'NONE',  ( 0.000000000000000000, 0.000000000000000000, -1.000000000000000000 ) ) ;
#87268=DIRECTION ( 'NONE',  ( -0.000000000000000000, 1.000000000000000000, -0.000000000000000000 ) ) ;
#87269=AXIS2_PLACEMENT_3D ( 'NONE', #93263, #23214, #31768 ) ;
#87270=DIRECTION ( 'NONE',  ( 0.000000000000000000, 0.000000000000000000, -1.000000000000000000 ) ) ;
#87271=DIRECTION ( 'NONE',  ( -4.274815082592931898E-19, -0.9999939076577903929, -0.003490651415223739937 ) ) ;
#87272=DIRECTION ( 'NONE',  ( 0.000000000000000000, -0.9999939076577903929, 0.003490651415223739937 ) ) ;
#87273=FACE_OUTER_BOUND ( 'NONE', #92280, .T. ) ;
#87274=AXIS2_PLACEMENT_3D ( 'NONE', #94539, #35009, #4861 ) ;
#87275=AXIS2_PLACEMENT_3D ( 'NONE', #60888, #70711, #10490 ) ;
#87276=DIRECTION ( 'NONE',  ( 0.000000000000000000, 1.000000000000000000, 0.000000000000000000 ) ) ;
#87278=EDGE_LOOP ( 'NONE', ( #58469, #65284, #61965, #56357 ) ) ;
#87279=ORIENTED_EDGE ( 'NONE', *, *, #109533, .F. ) ;
#87280=ORIENTED_EDGE ( 'NONE', *, *, #104818, .T. ) ;
#87281=FACE_OUTER_BOUND ( 'NONE', #127814, .T. ) ;
#87282=DIRECTION ( 'NONE',  ( 0.000000000000000000, 0.000000000000000000, -1.000000000000000000 ) ) ;
#87283=ORIENTED_EDGE ( 'NONE', *, *, #122745, .T. ) ;
#87285=VERTEX_POINT ( 'NONE', #123977 ) ;
#87286=DIRECTION ( 'NONE',  ( -0.000000000000000000, 1.000000000000000000, -0.000000000000000000 ) ) ;
#87287=AXIS2_PLACEMENT_3D ( 'NONE', #42883, #71664, #112886 ) ;
#87288=CONICAL_SURFACE ( 'NONE', #116534, 0.09999999999999982514, 0.003490658503988666988 ) ;
#87289=CIRCLE ( 'NONE', #53943, 0.09999999999999982514 ) ;
#87290=CARTESIAN_POINT ( 'NONE',  ( 2.499999999999947153, 2.500000000000000000, -3.637306695894650055 ) ) ;
#87291=DIRECTION ( 'NONE',  ( 0.000000000000000000, -0.000000000000000000, 1.000000000000000000 ) ) ;
#87292=DIRECTION ( 'NONE',  ( 0.000000000000000000, -0.9999939076577903929, 0.003490651415223739937 ) ) ;
#87293=CARTESIAN_POINT ( 'NONE',  ( -8.750000000000010658, 12.50000000000000000, -7.253104124594885960 ) ) ;
#87294=LINE ( 'NONE', #109534, #56996 ) ;
#87295=AXIS2_PLACEMENT_3D ( 'NONE', #33855, #4368, #114983 ) ;
#87296=VERTEX_POINT ( 'NONE', #34345 ) ;
#87297=DIRECTION ( 'NONE',  ( 0.000000000000000000, 0.000000000000000000, -1.000000000000000000 ) ) ;
#87298=ORIENTED_EDGE ( 'NONE', *, *, #22761, .F. ) ;
#87299=AXIS2_PLACEMENT_3D ( 'NONE', #210, #58526, #40165 ) ;
#87300=AXIS2_PLACEMENT_3D ( 'NONE', #17829, #5429, #66920 ) ;
#87301=ORIENTED_EDGE ( 'NONE', *, *, #44871, .F. ) ;
#87302=ORIENTED_EDGE ( 'NONE', *, *, #105736, .T. ) ;
#87303=DIRECTION ( 'NONE',  ( -4.274815082592931898E-19, -0.9999939076577903929, -0.003490651415223739937 ) ) ;
#87304=ORIENTED_EDGE ( 'NONE', *, *, #4366, .T. ) ;
#87305=ORIENTED_EDGE ( 'NONE', *, *, #96280, .T. ) ;
#87306=DIRECTION ( 'NONE',  ( 0.000000000000000000, 0.000000000000000000, -1.000000000000000000 ) ) ;
#87307=EDGE_CURVE ( 'NONE', #37082, #38247, #85723, .T. ) ;
#87308=CARTESIAN_POINT ( 'NONE',  ( 13.74999999999989697, 2.500000000000000000, 2.957883832488649389 ) ) ;
#87309=CARTESIAN_POINT ( 'NONE',  ( 15.39999999999989200, 12.50000000000000000, -0.6928203230275542523 ) ) ;
#87311=DIRECTION ( 'NONE',  ( 0.000000000000000000, 0.000000000000000000, -1.000000000000000000 ) ) ;
#87312=VECTOR ( 'NONE', #109154, 1000.000000000000000 ) ;
#87313=ORIENTED_EDGE ( 'NONE', *, *, #128714, .F. ) ;
#87314=CARTESIAN_POINT ( 'NONE',  ( 2.049999999999950084, 12.50000000000000000, 2.165063509461097713 ) ) ;
#87315=VERTEX_POINT ( 'NONE', #35618 ) ;
#87316=DIRECTION ( 'NONE',  ( 0.000000000000000000, 1.000000000000000000, 0.000000000000000000 ) ) ;
#87317=VERTEX_POINT ( 'NONE', #46081 ) ;
#87318=DIRECTION ( 'NONE',  ( 0.000000000000000000, 0.000000000000000000, 1.000000000000000000 ) ) ;
#87319=DIRECTION ( 'NONE',  ( -0.000000000000000000, -1.000000000000000000, -0.000000000000000000 ) ) ;
#87320=ORIENTED_EDGE ( 'NONE', *, *, #103970, .T. ) ;
#87321=CARTESIAN_POINT ( 'NONE',  ( -13.29999999999998828, 12.50000000000000000, 4.395220292106234439 ) ) ;
#87322=DIRECTION ( 'NONE',  ( 0.000000000000000000, -0.9999939076577903929, 0.003490651415223739937 ) ) ;
#87323=VERTEX_POINT ( 'NONE', #85975 ) ;
#87324=CIRCLE ( 'NONE', #70614, 0.1000000000000000472 ) ;
#87325=CIRCLE ( 'NONE', #104069, 0.06509327318403745899 ) ;
#87326=LINE ( 'NONE', #37613, #65400 ) ;
#87327=ORIENTED_EDGE ( 'NONE', *, *, #44201, .T. ) ;
#87328=VERTEX_POINT ( 'NONE', #114175 ) ;
#87329=DIRECTION ( 'NONE',  ( 0.000000000000000000, 1.000000000000000000, 0.000000000000000000 ) ) ;
#87330=FACE_OUTER_BOUND ( 'NONE', #106842, .T. ) ;
#87332=DIRECTION ( 'NONE',  ( 0.000000000000000000, 0.000000000000000000, -1.000000000000000000 ) ) ;
#87334=DIRECTION ( 'NONE',  ( 0.000000000000000000, 1.000000000000000000, 0.000000000000000000 ) ) ;
#87335=VECTOR ( 'NONE', #99053, 1000.000000000000000 ) ;
#87336=DIRECTION ( 'NONE',  ( 0.000000000000000000, 0.000000000000000000, 1.000000000000000000 ) ) ;
#87338=CARTESIAN_POINT ( 'NONE',  ( 6.449999999999931788, 2.500000000000000000, -2.411473670974877859 ) ) ;
#87339=CARTESIAN_POINT ( 'NONE',  ( 12.09999999999990550, 12.50000000000000000, -4.957854068765716882 ) ) ;
#87340=AXIS2_PLACEMENT_3D ( 'NONE', #86456, #28197, #7896 ) ;
#87341=ADVANCED_FACE ( 'NONE', ( #105646 ), #71068, .T. ) ;
#87342=ORIENTED_EDGE ( 'NONE', *, *, #77132, .T. ) ;
#87343=AXIS2_PLACEMENT_3D ( 'NONE', #102329, #51945, #61107 ) ;
#87344=EDGE_CURVE ( 'NONE', #9507, #20279, #54339, .T. ) ;
#87345=DIRECTION ( 'NONE',  ( 0.000000000000000000, 0.000000000000000000, 1.000000000000000000 ) ) ;
#87347=CARTESIAN_POINT ( 'NONE',  ( 1.899999999999951283, 12.50000000000000000, 0.2813168883297362810 ) ) ;
#87348=DIRECTION ( 'NONE',  ( 0.000000000000000000, 0.000000000000000000, 1.000000000000000000 ) ) ;
#87349=EDGE_CURVE ( 'NONE', #114894, #13624, #60621, .T. ) ;
#87350=DIRECTION ( 'NONE',  ( 0.000000000000000000, 0.000000000000000000, 1.000000000000000000 ) ) ;
#87351=VERTEX_POINT ( 'NONE', #39507 ) ;
#87352=CIRCLE ( 'NONE', #118664, 0.06509327318403745899 ) ;
#87353=DIRECTION ( 'NONE',  ( 0.000000000000000000, 0.000000000000000000, 1.000000000000000000 ) ) ;
#87354=DIRECTION ( 'NONE',  ( 0.000000000000000000, 1.000000000000000000, 0.000000000000000000 ) ) ;
#87355=AXIS2_PLACEMENT_3D ( 'NONE', #70890, #42749, #50591 ) ;
#87356=ADVANCED_FACE ( 'NONE', ( #48022 ), #79418, .T. ) ;
#87357=EDGE_CURVE ( 'NONE', #44082, #4682, #37631, .T. ) ;
#87358=EDGE_CURVE ( 'NONE', #119819, #107613, #123381, .T. ) ;
#87359=ADVANCED_FACE ( 'NONE', ( #87906 ), #41840, .T. ) ;
#87360=AXIS2_PLACEMENT_3D ( 'NONE', #4693, #42751, #114667 ) ;
#87361=VERTEX_POINT ( 'NONE', #17223 ) ;
#87362=VECTOR ( 'NONE', #46412, 1000.000000000000000 ) ;
#87363=FACE_OUTER_BOUND ( 'NONE', #62315, .T. ) ;
#87364=AXIS2_PLACEMENT_3D ( 'NONE', #33616, #34275, #93189 ) ;
#87365=ORIENTED_EDGE ( 'NONE', *, *, #58041, .T. ) ;
#87366=EDGE_LOOP ( 'NONE', ( #103830, #11499 ) ) ;
#87367=DIRECTION ( 'NONE',  ( -0.000000000000000000, -1.000000000000000000, -0.000000000000000000 ) ) ;
#87368=CIRCLE ( 'NONE', #62366, 0.1000000000000000472 ) ;
#87369=VERTEX_POINT ( 'NONE', #29659 ) ;
#87370=DIRECTION ( 'NONE',  ( 0.000000000000000000, 1.000000000000000000, 0.000000000000000000 ) ) ;
#87371=DIRECTION ( 'NONE',  ( -0.000000000000000000, -1.000000000000000000, -0.000000000000000000 ) ) ;
#87372=CIRCLE ( 'NONE', #76642, 0.06509327318403741736 ) ;
#87373=DIRECTION ( 'NONE',  ( 0.000000000000000000, 1.000000000000000000, 0.000000000000000000 ) ) ;
#87374=ORIENTED_EDGE ( 'NONE', *, *, #93356, .F. ) ;
#87375=FACE_BOUND ( 'NONE', #23890, .T. ) ;
#87376=DIRECTION ( 'NONE',  ( 0.000000000000000000, 0.000000000000000000, -1.000000000000000000 ) ) ;
#87377=ORIENTED_EDGE ( 'NONE', *, *, #14862, .F. ) ;
#87378=CARTESIAN_POINT ( 'NONE',  ( -1.050000000000038236, 12.50000000000000000, -1.818653347947326138 ) ) ;
#87379=VECTOR ( 'NONE', #1442, 1000.000000000000000 ) ;
#87380=CARTESIAN_POINT ( 'NONE',  ( 5.849999999999933031, 12.50000000000000000, 7.188010851410848723 ) ) ;
#87381=ORIENTED_EDGE ( 'NONE', *, *, #77977, .T. ) ;
#87382=CIRCLE ( 'NONE', #28926, 0.06509327318403745899 ) ;
#87383=AXIS2_PLACEMENT_3D ( 'NONE', #119251, #40060, #120550 ) ;
#87384=ORIENTED_EDGE ( 'NONE', *, *, #128105, .T. ) ;
#87385=ORIENTED_EDGE ( 'NONE', *, *, #544, .F. ) ;
#87386=CARTESIAN_POINT ( 'NONE',  ( -12.49999999999999467, 12.50000000000000000, 0.6928203230275535862 ) ) ;
#87387=CARTESIAN_POINT ( 'NONE',  ( -10.40000000000000213, 2.500000000000000000, 3.737306695894644371 ) ) ;
#87388=CARTESIAN_POINT ( 'NONE',  ( 11.04999999999990834, 2.500000000000000000, 1.818653347947321475 ) ) ;
#87389=EDGE_CURVE ( 'NONE', #34323, #128096, #69001, .T. ) ;
#87390=FACE_BOUND ( 'NONE', #109340, .T. ) ;
#87391=ORIENTED_EDGE ( 'NONE', *, *, #13925, .F. ) ;
#87393=CARTESIAN_POINT ( 'NONE',  ( 0.8499999999999527933, 2.500000000000000000, 7.288010851410849256 ) ) ;
#87394=EDGE_LOOP ( 'NONE', ( #18629, #73115, #106334, #103199 ) ) ;
#87395=DIRECTION ( 'NONE',  ( 0.000000000000000000, 0.000000000000000000, 1.000000000000000000 ) ) ;
#87396=PLANE ( 'NONE',  #86224 ) ;
#87397=EDGE_CURVE ( 'NONE', #53276, #108500, #76830, .T. ) ;
#87398=DIRECTION ( 'NONE',  ( 0.000000000000000000, 0.000000000000000000, 1.000000000000000000 ) ) ;
#87399=ADVANCED_FACE ( 'NONE', ( #127853 ), #109506, .T. ) ;
#87400=DIRECTION ( 'NONE',  ( 0.000000000000000000, 0.000000000000000000, 1.000000000000000000 ) ) ;
#87401=CARTESIAN_POINT ( 'NONE',  ( -7.500000000000016875, 12.50000000000000000, -3.702399969078687292 ) ) ;
#87402=EDGE_CURVE ( 'NONE', #109920, #79243, #119186, .T. ) ;
#87403=VERTEX_POINT ( 'NONE', #89220 ) ;
#87404=EDGE_LOOP ( 'NONE', ( #12143, #51732 ) ) ;
#87405=ORIENTED_EDGE ( 'NONE', *, *, #48692, .F. ) ;
#87406=AXIS2_PLACEMENT_3D ( 'NONE', #91637, #2593, #80542 ) ;
#87407=CONICAL_SURFACE ( 'NONE', #41487, 0.1000000000000000472, 0.003490658503988666988 ) ;
#87408=EDGE_LOOP ( 'NONE', ( #46915, #79013, #70423, #117710 ) ) ;
#87409=VERTEX_POINT ( 'NONE', #49323 ) ;
#87410=DIRECTION ( 'NONE',  ( -4.274815082592931898E-19, -0.9999939076577903929, -0.003490651415223739937 ) ) ;
#87411=EDGE_CURVE ( 'NONE', #2269, #86712, #118029, .T. ) ;
#87412=CARTESIAN_POINT ( 'NONE',  ( -7.100000000000018296, 2.500000000000000000, -4.330127018922201643 ) ) ;
#87413=ORIENTED_EDGE ( 'NONE', *, *, #82982, .F. ) ;
#87414=EDGE_CURVE ( 'NONE', #35299, #123030, #4142, .T. ) ;
#87415=FACE_BOUND ( 'NONE', #35820, .T. ) ;
#87416=DIRECTION ( 'NONE',  ( 0.000000000000000000, 0.000000000000000000, 1.000000000000000000 ) ) ;
#87417=EDGE_CURVE ( 'NONE', #41715, #112785, #98246, .T. ) ;
#87418=AXIS2_PLACEMENT_3D ( 'NONE', #9885, #99568, #49828 ) ;
#87419=EDGE_CURVE ( 'NONE', #72558, #110762, #97747, .T. ) ;
#87420=AXIS2_PLACEMENT_3D ( 'NONE', #92806, #12917, #103905 ) ;
#87421=ADVANCED_FACE ( 'NONE', ( #77464 ), #50239, .T. ) ;
#87422=CARTESIAN_POINT ( 'NONE',  ( -9.150000000000011013, 12.50000000000000000, -5.867463478539781896 ) ) ;
#87424=CARTESIAN_POINT ( 'NONE',  ( 13.34999999999989662, 2.500000000000000000, -2.957883832488653830 ) ) ;
#87425=CARTESIAN_POINT ( 'NONE',  ( 4.349999999999938360, 12.50000000000000000, 1.883746621131358934 ) ) ;
#87426=ORIENTED_EDGE ( 'NONE', *, *, #99415, .T. ) ;
#87427=DIRECTION ( 'NONE',  ( 0.000000000000000000, -0.000000000000000000, 1.000000000000000000 ) ) ;
#87428=EDGE_CURVE ( 'NONE', #3076, #92060, #121235, .T. ) ;
#87429=VERTEX_POINT ( 'NONE', #117355 ) ;
#87430=CIRCLE ( 'NONE', #68563, 0.06509327318403741736 ) ;
#87431=ORIENTED_EDGE ( 'NONE', *, *, #99197, .F. ) ;
#87432=ORIENTED_EDGE ( 'NONE', *, *, #39706, .F. ) ;
#87433=CARTESIAN_POINT ( 'NONE',  ( 5.649999999999932854, 2.500000000000000000, 1.718653347947321386 ) ) ;
#87434=CARTESIAN_POINT ( 'NONE',  ( 7.180215335565443446, 2.499999999999999112, 8.697219394475776966 ) ) ;
#87435=CARTESIAN_POINT ( 'NONE',  ( 1.849999999999951017, 12.50000000000000000, -6.213873640053564351 ) ) ;
#87436=VERTEX_POINT ( 'NONE', #126574 ) ;
#87437=CARTESIAN_POINT ( 'NONE',  ( 12.30568799110194611, 2.500000000000000000, -7.490555764795464810 ) ) ;
#87438=AXIS2_PLACEMENT_3D ( 'NONE', #75206, #63461, #32730 ) ;
#87439=CARTESIAN_POINT ( 'NONE',  ( -13.34999999999999076, 2.500000000000000000, 1.472243186433549456 ) ) ;
#87440=DIRECTION ( 'NONE',  ( 0.000000000000000000, 1.000000000000000000, 0.000000000000000000 ) ) ;
#87442=CARTESIAN_POINT ( 'NONE',  ( 7.699999999999925571, 12.50000000000000000, 3.918623584224382839 ) ) ;
#87443=DIRECTION ( 'NONE',  ( 0.000000000000000000, 0.000000000000000000, -1.000000000000000000 ) ) ;
#87444=CONICAL_SURFACE ( 'NONE', #24769, 0.09999999999999982514, 0.003490658503988666988 ) ;
#87445=DIRECTION ( 'NONE',  ( 0.000000000000000000, 0.000000000000000000, -1.000000000000000000 ) ) ;
#87446=ORIENTED_EDGE ( 'NONE', *, *, #5355, .T. ) ;
#87447=DIRECTION ( 'NONE',  ( 0.000000000000000000, 0.000000000000000000, -1.000000000000000000 ) ) ;
#87448=AXIS2_PLACEMENT_3D ( 'NONE', #56885, #120356, #10388 ) ;
#87449=VERTEX_POINT ( 'NONE', #27710 ) ;
#87450=ORIENTED_EDGE ( 'NONE', *, *, #91048, .F. ) ;
#87451=CARTESIAN_POINT ( 'NONE',  ( -1.450000000000035927, 12.50000000000000000, -1.818653347947326138 ) ) ;
#87452=CARTESIAN_POINT ( 'NONE',  ( -6.850000000000017408, 12.50000000000000000, -6.148780366869526226 ) ) ;
#87453=FACE_OUTER_BOUND ( 'NONE', #76958, .T. ) ;
#87454=EDGE_LOOP ( 'NONE', ( #95516, #80058 ) ) ;
#87455=ORIENTED_EDGE ( 'NONE', *, *, #83179, .F. ) ;
#87456=CARTESIAN_POINT ( 'NONE',  ( -6.250000000000015987, 2.500000000000000000, 1.472243186433545459 ) ) ;
#87457=AXIS2_PLACEMENT_3D ( 'NONE', #123743, #45214, #124415 ) ;
#87458=ADVANCED_FACE ( 'NONE', ( #8699 ), #35570, .T. ) ;
#87459=DIRECTION ( 'NONE',  ( 0.000000000000000000, 0.000000000000000000, -1.000000000000000000 ) ) ;
#87460=CARTESIAN_POINT ( 'NONE',  ( 11.04999999999991012, 2.500000000000000000, 6.841600689897072485 ) ) ;
#87461=EDGE_LOOP ( 'NONE', ( #100981, #103388 ) ) ;
#87462=VERTEX_POINT ( 'NONE', #60140 ) ;
#87463=FACE_OUTER_BOUND ( 'NONE', #118352, .T. ) ;
#87464=AXIS2_PLACEMENT_3D ( 'NONE', #106747, #17048, #85818 ) ;
#87465=VERTEX_POINT ( 'NONE', #20192 ) ;
#87466=DIRECTION ( 'NONE',  ( 0.000000000000000000, 0.000000000000000000, 1.000000000000000000 ) ) ;
#87467=CARTESIAN_POINT ( 'NONE',  ( 1.849999999999949685, 2.500000000000000000, -2.511473670974877948 ) ) ;
#87468=ORIENTED_EDGE ( 'NONE', *, *, #84640, .T. ) ;
#87469=DIRECTION ( 'NONE',  ( 0.000000000000000000, 0.000000000000000000, -1.000000000000000000 ) ) ;
#87470=CARTESIAN_POINT ( 'NONE',  ( -14.54999999999998472, 12.50000000000000000, -2.165063509461099489 ) ) ;
#87471=FACE_OUTER_BOUND ( 'NONE', #41060, .T. ) ;
#87472=CIRCLE ( 'NONE', #68699, 0.06509327318403745899 ) ;
#87473=EDGE_CURVE ( 'NONE', #26297, #81382, #56472, .T. ) ;
#87474=CARTESIAN_POINT ( 'NONE',  ( 4.799999999999939426, 2.500000000000000000, -4.776537180435977525 ) ) ;
#87475=ORIENTED_EDGE ( 'NONE', *, *, #45929, .F. ) ;
#87476=LINE ( 'NONE', #7629, #117849 ) ;
#87478=AXIS2_PLACEMENT_3D ( 'NONE', #26050, #36529, #95435 ) ;
#87479=VERTEX_POINT ( 'NONE', #21478 ) ;
#87480=VERTEX_POINT ( 'NONE', #111804 ) ;
#87481=PLANE ( 'NONE',  #37397 ) ;
#87482=DIRECTION ( 'NONE',  ( 0.000000000000000000, -0.000000000000000000, 1.000000000000000000 ) ) ;
#87483=CARTESIAN_POINT ( 'NONE',  ( 10.39999999999990976, 2.500000000000000000, -4.230127018922201998 ) ) ;
#87484=CARTESIAN_POINT ( 'NONE',  ( 9.349999999999916156, 2.500000000000000000, 6.048780366869520364 ) ) ;
#87485=CARTESIAN_POINT ( 'NONE',  ( -12.89999999999999147, 2.500000000000000000, -4.230127018922199333 ) ) ;
#87486=DIRECTION ( 'NONE',  ( -0.000000000000000000, -1.000000000000000000, -0.000000000000000000 ) ) ;
#87487=CARTESIAN_POINT ( 'NONE',  ( 10.84999999999991260, 12.50000000000000000, 7.188010851410848723 ) ) ;
#87488=DIRECTION ( 'NONE',  ( 0.000000000000000000, -0.9999939076577903929, 0.003490651415223739937 ) ) ;
#87489=DIRECTION ( 'NONE',  ( 0.000000000000000000, 1.000000000000000000, 0.000000000000000000 ) ) ;
#87490=CIRCLE ( 'NONE', #26866, 0.1000000000000002554 ) ;
#87491=CARTESIAN_POINT ( 'NONE',  ( -4.600000000000024514, 2.500000000000000000, -0.5928203230275542746 ) ) ;
#87492=AXIS2_PLACEMENT_3D ( 'NONE', #77854, #7824, #108610 ) ;
#87493=EDGE_CURVE ( 'NONE', #7181, #117167, #90196, .T. ) ;
#87494=AXIS2_PLACEMENT_3D ( 'NONE', #35994, #35352, #56265 ) ;
#87495=ORIENTED_EDGE ( 'NONE', *, *, #5373, .T. ) ;
#87496=CIRCLE ( 'NONE', #129310, 0.06509327318403745899 ) ;
#87497=DIRECTION ( 'NONE',  ( 0.000000000000000000, 1.000000000000000000, 0.000000000000000000 ) ) ;
#87498=CARTESIAN_POINT ( 'NONE',  ( 8.949999999999919353, 2.500000000000000000, 2.611473670974873151 ) ) ;
#87499=CARTESIAN_POINT ( 'NONE',  ( -2.100000000000033840, 2.500000000000000000, 4.922947341949748257 ) ) ;
#87500=FACE_OUTER_BOUND ( 'NONE', #10287, .T. ) ;
#87501=LINE ( 'NONE', #58074, #10304 ) ;
#87502=EDGE_CURVE ( 'NONE', #7687, #32088, #2088, .T. ) ;
#87503=CIRCLE ( 'NONE', #47827, 0.09999999999999982514 ) ;
#87504=VERTEX_POINT ( 'NONE', #110499 ) ;
#87505=CONICAL_SURFACE ( 'NONE', #127335, 0.1000000000000002554, 0.003490658503988666988 ) ;
#87506=CARTESIAN_POINT ( 'NONE',  ( -9.200000000000006395, 2.500000000000000000, 4.330127018922196314 ) ) ;
#87507=AXIS2_PLACEMENT_3D ( 'NONE', #27918, #68479, #67836 ) ;
#87508=AXIS2_PLACEMENT_3D ( 'NONE', #19842, #37552, #78115 ) ;
#87509=DIRECTION ( 'NONE',  ( 0.000000000000000000, 0.000000000000000000, 1.000000000000000000 ) ) ;
#87510=CARTESIAN_POINT ( 'NONE',  ( -0.4500000000000402012, 12.50000000000000000, 6.495190528383297135 ) ) ;
#87511=ORIENTED_EDGE ( 'NONE', *, *, #123228, .T. ) ;
#87512=EDGE_CURVE ( 'NONE', #63031, #6029, #94139, .T. ) ;
#87514=EDGE_CURVE ( 'NONE', #76556, #42141, #106737, .T. ) ;
#87515=EDGE_CURVE ( 'NONE', #120954, #87216, #90011, .T. ) ;
#87516=EDGE_CURVE ( 'NONE', #70542, #126334, #39217, .T. ) ;
#87517=AXIS2_PLACEMENT_3D ( 'NONE', #15418, #55369, #5594 ) ;
#87518=ORIENTED_EDGE ( 'NONE', *, *, #25621, .F. ) ;
#87519=CIRCLE ( 'NONE', #64543, 0.09999999999999999167 ) ;
#87520=EDGE_LOOP ( 'NONE', ( #100982, #14456, #47893, #67932 ) ) ;
#87521=ORIENTED_EDGE ( 'NONE', *, *, #108820, .T. ) ;
#87522=ORIENTED_EDGE ( 'NONE', *, *, #50687, .T. ) ;
#87524=EDGE_CURVE ( 'NONE', #79569, #95487, #71149, .T. ) ;
#87525=FACE_OUTER_BOUND ( 'NONE', #6452, .T. ) ;
#87526=CARTESIAN_POINT ( 'NONE',  ( -9.350000000000008527, 2.500000000000000000, -6.148780366869520897 ) ) ;
#87527=EDGE_CURVE ( 'NONE', #13366, #63398, #1827, .T. ) ;
#87528=FACE_OUTER_BOUND ( 'NONE', #8861, .T. ) ;
#87529=AXIS2_PLACEMENT_3D ( 'NONE', #65714, #14665, #104357 ) ;
#87530=EDGE_CURVE ( 'NONE', #86533, #2794, #110852, .T. ) ;
#87531=EDGE_LOOP ( 'NONE', ( #127857, #89711 ) ) ;
#87532=B_SPLINE_CURVE_WITH_KNOTS ( 'NONE', 3,
 ( #56522, #18537, #76178, #116094 ),
 .UNSPECIFIED., .F., .F.,
 ( 4, 4 ),
 ( 8.673617379884035472E-19, 0.002128161363186473892 ),
 .UNSPECIFIED. ) ;
#87533=CARTESIAN_POINT ( 'NONE',  ( 3.149999999999942624, 2.500000000000000000, 6.048780366869521252 ) ) ;
#87534=ORIENTED_EDGE ( 'NONE', *, *, #86177, .T. ) ;
#87535=VECTOR ( 'NONE', #26671, 1000.000000000000000 ) ;
#87536=CARTESIAN_POINT ( 'NONE',  ( 35.04009662971161276, -1.562391656609272594, -4.793251516055618389 ) ) ;
#87537=DIRECTION ( 'NONE',  ( 0.000000000000000000, -0.9999939076577903929, 0.003490651415223739937 ) ) ;
#87538=CARTESIAN_POINT ( 'NONE',  ( 12.49999999999990052, 2.500000000000000000, 0.7928203230275495672 ) ) ;
#87539=CARTESIAN_POINT ( 'NONE',  ( -6.700000000000016165, 2.500000000000000000, 4.230127018922196669 ) ) ;
#87540=CARTESIAN_POINT ( 'NONE',  ( -12.09999999999999609, 2.500000000000000000, 4.430127018922196847 ) ) ;
#87541=VERTEX_POINT ( 'NONE', #99405 ) ;
#87542=AXIS2_PLACEMENT_3D ( 'NONE', #114860, #23928, #113590 ) ;
#87543=EDGE_LOOP ( 'NONE', ( #118838, #89509, #129247, #57865 ) ) ;
#87544=ORIENTED_EDGE ( 'NONE', *, *, #82991, .T. ) ;
#87545=ORIENTED_EDGE ( 'NONE', *, *, #64687, .F. ) ;
#87546=DIRECTION ( 'NONE',  ( 0.000000000000000000, 0.000000000000000000, 1.000000000000000000 ) ) ;
#87547=CARTESIAN_POINT ( 'NONE',  ( 1.849999999999949685, 2.500000000000000000, 1.818653347947321475 ) ) ;
#87548=DIRECTION ( 'NONE',  ( 0.000000000000000000, 0.000000000000000000, 1.000000000000000000 ) ) ;
#87549=FACE_BOUND ( 'NONE', #78947, .T. ) ;
#87550=DIRECTION ( 'NONE',  ( 0.000000000000000000, 0.000000000000000000, 1.000000000000000000 ) ) ;
#87551=DIRECTION ( 'NONE',  ( 0.000000000000000000, 0.000000000000000000, -1.000000000000000000 ) ) ;
#87552=CIRCLE ( 'NONE', #29096, 0.06509327318403745899 ) ;
#87553=DIRECTION ( 'NONE',  ( -0.000000000000000000, -1.000000000000000000, -0.000000000000000000 ) ) ;
#87554=LINE ( 'NONE', #35890, #60408 ) ;
#87557=PLANE ( 'NONE',  #113670 ) ;
#87558=AXIS2_PLACEMENT_3D ( 'NONE', #12109, #11470, #31769 ) ;
#87559=DIRECTION ( 'NONE',  ( 0.000000000000000000, 1.000000000000000000, 0.000000000000000000 ) ) ;
#87560=CARTESIAN_POINT ( 'NONE',  ( 7.699999999999923794, 2.500000000000000000, 4.776537180435972196 ) ) ;
#87561=AXIS2_PLACEMENT_3D ( 'NONE', #119230, #120526, #29561 ) ;
#87562=EDGE_LOOP ( 'NONE', ( #54139, #68237, #57770, #97008 ) ) ;
#87563=VERTEX_POINT ( 'NONE', #100664 ) ;
#87564=EDGE_LOOP ( 'NONE', ( #42841, #26738, #75667, #52018 ) ) ;
#87565=VERTEX_POINT ( 'NONE', #100044 ) ;
#87566=VECTOR ( 'NONE', #118823, 1000.000000000000000 ) ;
#87567=FACE_OUTER_BOUND ( 'NONE', #97804, .T. ) ;
#87568=EDGE_CURVE ( 'NONE', #120419, #20260, #9728, .T. ) ;
#87569=FACE_BOUND ( 'NONE', #108327, .T. ) ;
#87570=FACE_OUTER_BOUND ( 'NONE', #56168, .T. ) ;
#87571=EDGE_CURVE ( 'NONE', #79978, #4381, #123462, .T. ) ;
#87572=CIRCLE ( 'NONE', #79288, 0.1000000000000000472 ) ;
#87573=AXIS2_PLACEMENT_3D ( 'NONE', #111697, #53428, #33145 ) ;
#87574=ADVANCED_FACE ( 'NONE', ( #1190 ), #41142, .T. ) ;
#87575=VERTEX_POINT ( 'NONE', #51599 ) ;
#87576=PLANE ( 'NONE',  #36278 ) ;
#87577=CARTESIAN_POINT ( 'NONE',  ( 7.899999999999924860, 12.50000000000000000, -4.330127018922201643 ) ) ;
#87578=CARTESIAN_POINT ( 'NONE',  ( -6.450000000000016165, 12.50000000000000000, 2.576566944158910744 ) ) ;
#87579=ORIENTED_EDGE ( 'NONE', *, *, #125485, .F. ) ;
#87580=DIRECTION ( 'NONE',  ( 0.000000000000000000, 0.000000000000000000, 1.000000000000000000 ) ) ;
#87581=DIRECTION ( 'NONE',  ( -0.000000000000000000, 1.000000000000000000, -0.000000000000000000 ) ) ;
#87582=ADVANCED_FACE ( 'NONE', ( #81682 ), #37714, .T. ) ;
#87583=VERTEX_POINT ( 'NONE', #88933 ) ;
#87584=AXIS2_PLACEMENT_3D ( 'NONE', #14943, #54897, #94831 ) ;
#87585=DIRECTION ( 'NONE',  ( 0.000000000000000000, 0.000000000000000000, -1.000000000000000000 ) ) ;
#87586=LINE ( 'NONE', #117031, #70604 ) ;
#87587=ORIENTED_EDGE ( 'NONE', *, *, #83944, .T. ) ;
#87588=AXIS2_PLACEMENT_3D ( 'NONE', #118429, #98784, #69988 ) ;
#87589=CARTESIAN_POINT ( 'NONE',  ( 10.59999999999991260, 12.50000000000000000, 0.2813168883297361700 ) ) ;
#87590=AXIS2_PLACEMENT_3D ( 'NONE', #7807, #108593, #118410 ) ;
#87591=DIRECTION ( 'NONE',  ( 0.000000000000000000, 0.000000000000000000, 1.000000000000000000 ) ) ;
#87592=ORIENTED_EDGE ( 'NONE', *, *, #115542, .F. ) ;
#87593=DIRECTION ( 'NONE',  ( 0.000000000000000000, -0.9999939076577903929, 0.003490651415223739937 ) ) ;
#87594=ORIENTED_EDGE ( 'NONE', *, *, #95668, .T. ) ;
#87596=FACE_OUTER_BOUND ( 'NONE', #98336, .T. ) ;
#87597=EDGE_CURVE ( 'NONE', #68741, #28244, #67021, .T. ) ;
#87598=CONICAL_SURFACE ( 'NONE', #35302, 0.1000000000000000472, 0.003490658503988666988 ) ;
#87599=EDGE_LOOP ( 'NONE', ( #49946, #33565, #92713, #40088 ) ) ;
#87600=CARTESIAN_POINT ( 'NONE',  ( -1.050000000000038236, 12.50000000000000000, -1.818653347947326138 ) ) ;
#87601=FACE_BOUND ( 'NONE', #36066, .T. ) ;
#87602=CONICAL_SURFACE ( 'NONE', #79318, 0.1000000000000002554, 0.003490658503988666988 ) ;
#87603=AXIS2_PLACEMENT_3D ( 'NONE', #39362, #9876, #120470 ) ;
#87605=CARTESIAN_POINT ( 'NONE',  ( -3.350000000000028955, 12.50000000000000000, 5.867463478539781896 ) ) ;
#87606=ORIENTED_EDGE ( 'NONE', *, *, #72772, .T. ) ;
#87607=LINE ( 'NONE', #96774, #85893 ) ;
#87608=DIRECTION ( 'NONE',  ( -4.274815082592931898E-19, -0.9999939076577903929, -0.003490651415223739937 ) ) ;
#87609=CARTESIAN_POINT ( 'NONE',  ( -3.749999999999991118, 12.50000000000000000, 2.230156782645134950 ) ) ;
#87610=CARTESIAN_POINT ( 'NONE',  ( -8.350000000000012079, 2.500000000000000000, 2.957883832488649389 ) ) ;
#87611=CARTESIAN_POINT ( 'NONE',  ( 17.50000000000011013, 2.362783583789868302, -3.757116699121217707 ) ) ;
#87612=CIRCLE ( 'NONE', #56406, 0.06509327318403745899 ) ;
#87613=EDGE_LOOP ( 'NONE', ( #93219, #91758, #45577, #126557 ) ) ;
#87614=ORIENTED_EDGE ( 'NONE', *, *, #3861, .T. ) ;
#87615=FACE_OUTER_BOUND ( 'NONE', #63598, .T. ) ;
#87616=EDGE_CURVE ( 'NONE', #76977, #84673, #29404, .T. ) ;
#87617=LINE ( 'NONE', #86979, #112083 ) ;
#87618=CARTESIAN_POINT ( 'NONE',  ( -2.950000000000033484, 12.50000000000000000, -6.430097255199264339 ) ) ;
#87619=ORIENTED_EDGE ( 'NONE', *, *, #6252, .F. ) ;
#87620=EDGE_LOOP ( 'NONE', ( #28937, #29552, #12139, #35995 ) ) ;
#87621=ORIENTED_EDGE ( 'NONE', *, *, #51964, .T. ) ;
#87622=CARTESIAN_POINT ( 'NONE',  ( -5.850000000000018296, 12.50000000000000000, 2.792790559304612064 ) ) ;
#87623=DIRECTION ( 'NONE',  ( -0.000000000000000000, 1.000000000000000000, -0.000000000000000000 ) ) ;
#87625=CARTESIAN_POINT ( 'NONE',  ( 1.049999999999954525, 2.500000000000000000, -2.511473670974877948 ) ) ;
#87626=DIRECTION ( 'NONE',  ( 0.000000000000000000, 0.000000000000000000, 1.000000000000000000 ) ) ;
#87627=DIRECTION ( 'NONE',  ( -4.274815082592931898E-19, -0.9999939076577903929, -0.003490651415223739937 ) ) ;
#87629=CIRCLE ( 'NONE', #39645, 0.09999999999999982514 ) ;
#87630=DIRECTION ( 'NONE',  ( 0.000000000000000000, 1.000000000000000000, 0.000000000000000000 ) ) ;
#87631=EDGE_CURVE ( 'NONE', #15166, #103763, #81611, .T. ) ;
#87633=VERTEX_POINT ( 'NONE', #33254 ) ;
#87634=ORIENTED_EDGE ( 'NONE', *, *, #104727, .F. ) ;
#87635=CARTESIAN_POINT ( 'NONE',  ( 3.349999999999941913, 12.50000000000000000, 6.495190528383297135 ) ) ;
#87637=EDGE_LOOP ( 'NONE', ( #56859, #3126 ) ) ;
#87638=ORIENTED_EDGE ( 'NONE', *, *, #64625, .T. ) ;
#87639=DIRECTION ( 'NONE',  ( 0.000000000000000000, 0.000000000000000000, 1.000000000000000000 ) ) ;
#87640=CARTESIAN_POINT ( 'NONE',  ( -13.34999999999999076, 2.500000000000000000, -2.065063509461099844 ) ) ;
#87641=AXIS2_PLACEMENT_3D ( 'NONE', #123856, #74136, #42098 ) ;
#87642=CARTESIAN_POINT ( 'NONE',  ( -5.850000000000018296, 2.500000000000000000, 7.188010851410848723 ) ) ;
#87644=CARTESIAN_POINT ( 'NONE',  ( -3.950000000000025491, 2.500000000000000000, 6.148780366869520897 ) ) ;
#87645=FACE_OUTER_BOUND ( 'NONE', #82962, .T. ) ;
#87646=DIRECTION ( 'NONE',  ( -4.274815082592931898E-19, -0.9999939076577903929, -0.003490651415223739937 ) ) ;
#87647=ORIENTED_EDGE ( 'NONE', *, *, #86853, .F. ) ;
#87648=LINE ( 'NONE', #87013, #36851 ) ;
#87649=AXIS2_PLACEMENT_3D ( 'NONE', #17908, #78795, #87291 ) ;
#87650=DIRECTION ( 'NONE',  ( 0.000000000000000000, 1.000000000000000000, 0.000000000000000000 ) ) ;
#87651=ORIENTED_EDGE ( 'NONE', *, *, #22918, .T. ) ;
#87652=EDGE_CURVE ( 'NONE', #126997, #24357, #35183, .T. ) ;
#87653=CIRCLE ( 'NONE', #102346, 0.1000000000000000472 ) ;
#87654=AXIS2_PLACEMENT_3D ( 'NONE', #6389, #116369, #46341 ) ;
#87655=ORIENTED_EDGE ( 'NONE', *, *, #91665, .T. ) ;
#87656=CIRCLE ( 'NONE', #10394, 0.06509327318403745899 ) ;
#87657=VERTEX_POINT ( 'NONE', #52877 ) ;
#87658=VERTEX_POINT ( 'NONE', #22790 ) ;
#87659=DIRECTION ( 'NONE',  ( 0.000000000000000000, 0.000000000000000000, -1.000000000000000000 ) ) ;
#87660=DIRECTION ( 'NONE',  ( 0.000000000000000000, -0.9999939076577903929, 0.003490651415223739937 ) ) ;
#87661=EDGE_CURVE ( 'NONE', #59275, #62448, #100489, .T. ) ;
#87662=AXIS2_PLACEMENT_3D ( 'NONE', #109049, #80912, #10236 ) ;
#87663=CONICAL_SURFACE ( 'NONE', #31259, 0.09999999999999982514, 0.003490658503988666988 ) ;
#87664=ORIENTED_EDGE ( 'NONE', *, *, #43518, .T. ) ;
#87665=LINE ( 'NONE', #36666, #65216 ) ;
#87666=CARTESIAN_POINT ( 'NONE',  ( -4.800000000000028244, 2.500000000000000000, -3.983716857408426293 ) ) ;
#87667=ORIENTED_EDGE ( 'NONE', *, *, #87414, .T. ) ;
#87668=ADVANCED_FACE ( 'NONE', ( #24063 ), #75091, .T. ) ;
#87669=ADVANCED_FACE ( 'NONE', ( #114994 ), #72527, .T. ) ;
#87670=ADVANCED_FACE ( 'NONE', ( #12921 ), #62705, .T. ) ;
#87671=CARTESIAN_POINT ( 'NONE',  ( -13.54999999999999005, 12.50000000000000000, 2.576566944158914740 ) ) ;
#87672=EDGE_CURVE ( 'NONE', #97290, #3112, #102606, .T. ) ;
#87673=DIRECTION ( 'NONE',  ( 0.000000000000000000, 0.000000000000000000, 1.000000000000000000 ) ) ;
#87674=EDGE_LOOP ( 'NONE', ( #69721, #77518 ) ) ;
#87675=EDGE_LOOP ( 'NONE', ( #54281, #35860 ) ) ;
#87676=ADVANCED_FACE ( 'NONE', ( #14846 ), #87860, .T. ) ;
#87677=ORIENTED_EDGE ( 'NONE', *, *, #118219, .F. ) ;
#87678=AXIS2_PLACEMENT_3D ( 'NONE', #1615, #122690, #101767 ) ;
#87679=PLANE ( 'NONE',  #92699 ) ;
#87680=ADVANCED_FACE ( 'NONE', ( #124193 ), #3136, .T. ) ;
#87681=EDGE_CURVE ( 'NONE', #33854, #58766, #31459, .T. ) ;
#87682=DIRECTION ( 'NONE',  ( 0.000000000000000000, 1.000000000000000000, 0.000000000000000000 ) ) ;
#87683=EDGE_CURVE ( 'NONE', #61095, #113875, #5045, .T. ) ;
#87684=CIRCLE ( 'NONE', #83508, 0.09999999999999982514 ) ;
#87685=ADVANCED_FACE ( 'NONE', ( #43722 ), #35656, .T. ) ;
#87686=CIRCLE ( 'NONE', #75177, 0.06509327318403745899 ) ;
#87687=ORIENTED_EDGE ( 'NONE', *, *, #19094, .T. ) ;
#87688=CARTESIAN_POINT ( 'NONE',  ( -6.250000000000021316, 2.500000000000000000, -1.472243186433550122 ) ) ;
#87689=DIRECTION ( 'NONE',  ( -0.000000000000000000, 1.000000000000000000, -0.000000000000000000 ) ) ;
#87690=CARTESIAN_POINT ( 'NONE',  ( 6.649999999999931966, 2.500000000000000000, -7.088010851410853519 ) ) ;
#87691=CARTESIAN_POINT ( 'NONE',  ( 4.799999999999939426, 12.50000000000000000, -4.741630453620015118 ) ) ;
#87692=EDGE_CURVE ( 'NONE', #73692, #2801, #94086, .T. ) ;
#87693=CONICAL_SURFACE ( 'NONE', #104426, 0.1000000000000002554, 0.003490658503988666988 ) ;
#87694=VECTOR ( 'NONE', #32925, 1000.000000000000000 ) ;
#87696=CARTESIAN_POINT ( 'NONE',  ( 8.749999999999953815, 2.500000000000000000, 6.495190528383297135 ) ) ;
#87698=VERTEX_POINT ( 'NONE', #114362 ) ;
#87699=DIRECTION ( 'NONE',  ( 0.000000000000000000, 0.000000000000000000, -1.000000000000000000 ) ) ;
#87700=FACE_OUTER_BOUND ( 'NONE', #55840, .T. ) ;
#87701=FACE_BOUND ( 'NONE', #34680, .T. ) ;
#87702=AXIS2_PLACEMENT_3D ( 'NONE', #61668, #120576, #59748 ) ;
#87703=CARTESIAN_POINT ( 'NONE',  ( -5.400000000000019895, 2.500000000000000000, -2.276824562219559311E-15 ) ) ;
#87704=DIRECTION ( 'NONE',  ( 0.000000000000000000, 0.000000000000000000, 1.000000000000000000 ) ) ;
#87705=DIRECTION ( 'NONE',  ( 0.000000000000000000, 1.000000000000000000, 0.000000000000000000 ) ) ;
#87707=ORIENTED_EDGE ( 'NONE', *, *, #98179, .F. ) ;
#87708=CARTESIAN_POINT ( 'NONE',  ( -16.50000000000000000, 2.500000000000000000, 1.734723475976807094E-15 ) ) ;
#87709=DIRECTION ( 'NONE',  ( -0.000000000000000000, 1.000000000000000000, -0.000000000000000000 ) ) ;
#87710=CARTESIAN_POINT ( 'NONE',  ( -6.450000000000016165, 12.50000000000000000, 6.841600689897072485 ) ) ;
#87711=CARTESIAN_POINT ( 'NONE',  ( 6.049999999999932321, 12.50000000000000000, 6.906693963081109722 ) ) ;
#87712=ORIENTED_EDGE ( 'NONE', *, *, #11830, .F. ) ;
#87713=CARTESIAN_POINT ( 'NONE',  ( 3.749999999999938716, 2.500000000000000000, 7.188010851410848723 ) ) ;
#87714=DIRECTION ( 'NONE',  ( 0.000000000000000000, -0.9999939076577903929, 0.003490651415223739937 ) ) ;
#87715=CIRCLE ( 'NONE', #129615, 0.06509327318403745899 ) ;
#87716=VERTEX_POINT ( 'NONE', #63338 ) ;
#87717=ORIENTED_EDGE ( 'NONE', *, *, #84258, .F. ) ;
#87718=CARTESIAN_POINT ( 'NONE',  ( -5.650000000000023448, 2.500000000000000000, -1.818653347947326138 ) ) ;
#87719=CARTESIAN_POINT ( 'NONE',  ( 12.89999999999990266, 2.500000000000000000, -5.022947341949754119 ) ) ;
#87720=FACE_BOUND ( 'NONE', #2493, .T. ) ;
#87721=DIRECTION ( 'NONE',  ( 0.000000000000000000, 1.000000000000000000, 0.000000000000000000 ) ) ;
#87722=ADVANCED_FACE ( 'NONE', ( #103270 ), #127, .T. ) ;
#87723=ORIENTED_EDGE ( 'NONE', *, *, #58613, .F. ) ;
#87724=DIRECTION ( 'NONE',  ( 0.000000000000000000, 0.000000000000000000, 1.000000000000000000 ) ) ;
#87725=ADVANCED_FACE ( 'NONE', ( #34545 ), #62843, .T. ) ;
#87726=ORIENTED_EDGE ( 'NONE', *, *, #81293, .F. ) ;
#87727=ORIENTED_EDGE ( 'NONE', *, *, #64001, .F. ) ;
#87728=FACE_OUTER_BOUND ( 'NONE', #4725, .T. ) ;
#87730=ORIENTED_EDGE ( 'NONE', *, *, #47624, .F. ) ;
#87731=CARTESIAN_POINT ( 'NONE',  ( -12.89999999999999147, 12.50000000000000000, -0.7579135962115874925 ) ) ;
#87732=CARTESIAN_POINT ( 'NONE',  ( 9.999999999999916511, 2.500000000000000000, -0.6928203230275541413 ) ) ;
#87733=EDGE_CURVE ( 'NONE', #47201, #98668, #113008, .T. ) ;
#87734=CARTESIAN_POINT ( 'NONE',  ( 3.749999999999975131, 2.500000000000000000, 6.495190528383297135 ) ) ;
#87735=AXIS2_PLACEMENT_3D ( 'NONE', #31944, #33243, #92126 ) ;
#87736=LINE ( 'NONE', #59612, #17523 ) ;
#87737=ORIENTED_EDGE ( 'NONE', *, *, #120909, .F. ) ;
#87738=CARTESIAN_POINT ( 'NONE',  ( 9.999999999999912959, 12.50000000000000000, 3.572213422710607489 ) ) ;
#87739=CONICAL_SURFACE ( 'NONE', #50126, 0.1000000000000002554, 0.003490658503988666988 ) ;
#87740=CONICAL_SURFACE ( 'NONE', #60595, 0.1000000000000002554, 0.003490658503988666988 ) ;
#87741=CARTESIAN_POINT ( 'NONE',  ( 12.29999999999990479, 2.500000000000000000, 4.676537180435972552 ) ) ;
#87742=CARTESIAN_POINT ( 'NONE',  ( -11.44999999999999751, 12.50000000000000000, -6.906693963081111498 ) ) ;
#87743=DIRECTION ( 'NONE',  ( -0.000000000000000000, 1.000000000000000000, -0.000000000000000000 ) ) ;
#87744=VECTOR ( 'NONE', #107567, 1000.000000000000000 ) ;
#87745=ORIENTED_EDGE ( 'NONE', *, *, #28870, .T. ) ;
#87746=LINE ( 'NONE', #20799, #35015 ) ;
#87747=ORIENTED_EDGE ( 'NONE', *, *, #38543, .T. ) ;
#87748=DIRECTION ( 'NONE',  ( 0.000000000000000000, 0.000000000000000000, 1.000000000000000000 ) ) ;
#87749=ORIENTED_EDGE ( 'NONE', *, *, #59949, .F. ) ;
#87750=DIRECTION ( 'NONE',  ( 0.000000000000000000, 1.000000000000000000, 0.000000000000000000 ) ) ;
#87751=AXIS2_PLACEMENT_3D ( 'NONE', #2835, #42793, #82703 ) ;
#87752=AXIS2_PLACEMENT_3D ( 'NONE', #128958, #26865, #58908 ) ;
#87753=CARTESIAN_POINT ( 'NONE',  ( 17.50000000000000000, -2.499999999999999556, 2.666666666666670515 ) ) ;
#87754=DIRECTION ( 'NONE',  ( 0.000000000000000000, 0.000000000000000000, 1.000000000000000000 ) ) ;
#87755=DIRECTION ( 'NONE',  ( 0.000000000000000000, -0.000000000000000000, 1.000000000000000000 ) ) ;
#87756=EDGE_LOOP ( 'NONE', ( #99547, #24154, #68998, #46844 ) ) ;
#87757=LINE ( 'NONE', #9209, #18227 ) ;
#87758=CARTESIAN_POINT ( 'NONE',  ( 10.79999999999991012, 2.500000000000000000, -4.330127018922201643 ) ) ;
#87759=DIRECTION ( 'NONE',  ( 0.000000000000000000, 0.000000000000000000, 1.000000000000000000 ) ) ;
#87760=CARTESIAN_POINT ( 'NONE',  ( 0.8499999999999557909, 12.50000000000000000, -7.188010851410854052 ) ) ;
#87761=LINE ( 'NONE', #48498, #112194 ) ;
#87762=EDGE_CURVE ( 'NONE', #58821, #58767, #116285, .T. ) ;
#87763=ORIENTED_EDGE ( 'NONE', *, *, #100698, .T. ) ;
#87764=ORIENTED_EDGE ( 'NONE', *, *, #43979, .F. ) ;
#87765=DIRECTION ( 'NONE',  ( 0.000000000000000000, 0.000000000000000000, -1.000000000000000000 ) ) ;
#87766=ORIENTED_EDGE ( 'NONE', *, *, #24840, .T. ) ;
#87767=DIRECTION ( 'NONE',  ( 0.000000000000000000, -0.9999939076577903929, 0.003490651415223739937 ) ) ;
#87768=VERTEX_POINT ( 'NONE', #96018 ) ;
#87769=ORIENTED_EDGE ( 'NONE', *, *, #39887, .F. ) ;
#87770=ORIENTED_EDGE ( 'NONE', *, *, #123422, .T. ) ;
#87771=DIRECTION ( 'NONE',  ( 0.000000000000000000, -0.000000000000000000, 1.000000000000000000 ) ) ;
#87772=CONICAL_SURFACE ( 'NONE', #106556, 0.1000000000000000056, 0.003490658503988666988 ) ;
#87773=DIRECTION ( 'NONE',  ( 0.000000000000000000, 1.000000000000000000, 0.000000000000000000 ) ) ;
#87774=CIRCLE ( 'NONE', #33514, 0.06509327318403745899 ) ;
#87775=CARTESIAN_POINT ( 'NONE',  ( 3.749999999999978684, 12.50000000000000000, -2.165063509461101710 ) ) ;
#87776=CARTESIAN_POINT ( 'NONE',  ( -7.300000000000018474, 2.500000000000000000, -3.983716857408426293 ) ) ;
#87777=DIRECTION ( 'NONE',  ( 0.000000000000000000, -0.9999939076577903929, 0.003490651415223739937 ) ) ;
#87778=EDGE_CURVE ( 'NONE', #59465, #125538, #65248, .T. ) ;
#87779=CARTESIAN_POINT ( 'NONE',  ( 14.19999999999989626, 2.500000000000000000, -2.276824562219559311E-15 ) ) ;
#87780=LINE ( 'NONE', #4867, #36370 ) ;
#87781=ADVANCED_FACE ( 'NONE', ( #65904 ), #85806, .T. ) ;
#87782=DIRECTION ( 'NONE',  ( 0.000000000000000000, 0.000000000000000000, 1.000000000000000000 ) ) ;
#87783=AXIS2_PLACEMENT_3D ( 'NONE', #85606, #125529, #35872 ) ;
#87784=ORIENTED_EDGE ( 'NONE', *, *, #5693, .F. ) ;
#87785=ORIENTED_EDGE ( 'NONE', *, *, #8627, .T. ) ;
#87786=VERTEX_POINT ( 'NONE', #26000 ) ;
#87787=ORIENTED_EDGE ( 'NONE', *, *, #81441, .F. ) ;
#87788=DIRECTION ( 'NONE',  ( -0.000000000000000000, -1.000000000000000000, -0.000000000000000000 ) ) ;
#87789=ORIENTED_EDGE ( 'NONE', *, *, #116613, .T. ) ;
#87790=ADVANCED_FACE ( 'NONE', ( #105187 ), #88098, .T. ) ;
#87791=EDGE_LOOP ( 'NONE', ( #38663, #112908, #123107, #6402 ) ) ;
#87792=VECTOR ( 'NONE', #120274, 1000.000000000000000 ) ;
#87793=CIRCLE ( 'NONE', #16674, 0.1000000000000000472 ) ;
#87794=DIRECTION ( 'NONE',  ( 0.000000000000000000, 1.000000000000000000, 0.000000000000000000 ) ) ;
#87795=DIRECTION ( 'NONE',  ( 0.000000000000000000, 0.000000000000000000, -1.000000000000000000 ) ) ;
#87796=CIRCLE ( 'NONE', #31395, 0.1000000000000000472 ) ;
#87797=CARTESIAN_POINT ( 'NONE',  ( -10.00000000000000355, 2.500000000000000000, -0.5928203230275541635 ) ) ;
#87798=DIRECTION ( 'NONE',  ( -0.000000000000000000, -1.000000000000000000, -0.000000000000000000 ) ) ;
#87799=DIRECTION ( 'NONE',  ( 0.000000000000000000, 0.000000000000000000, -1.000000000000000000 ) ) ;
#87800=ORIENTED_EDGE ( 'NONE', *, *, #48262, .F. ) ;
#87801=CARTESIAN_POINT ( 'NONE',  ( -0.6500000000000394351, 2.500000000000000000, 2.611473670974873151 ) ) ;
#87802=AXIS2_PLACEMENT_3D ( 'NONE', #75307, #7199, #115203 ) ;
#87803=VERTEX_POINT ( 'NONE', #27921 ) ;
#87804=DIRECTION ( 'NONE',  ( -0.000000000000000000, 1.000000000000000000, -0.000000000000000000 ) ) ;
#87805=ORIENTED_EDGE ( 'NONE', *, *, #106790, .F. ) ;
#87806=CARTESIAN_POINT ( 'NONE',  ( 10.84999999999990905, 2.500000000000000000, 1.572243186433545548 ) ) ;
#87807=CIRCLE ( 'NONE', #104551, 0.1000000000000000472 ) ;
#87808=VERTEX_POINT ( 'NONE', #115643 ) ;
#87809=VERTEX_POINT ( 'NONE', #8269 ) ;
#87810=PLANE ( 'NONE',  #56562 ) ;
#87811=DIRECTION ( 'NONE',  ( -0.000000000000000000, -1.000000000000000000, -0.000000000000000000 ) ) ;
#87812=ADVANCED_FACE ( 'NONE', ( #16141 ), #126774, .T. ) ;
#87813=CARTESIAN_POINT ( 'NONE',  ( -13.34999999999999076, 12.50000000000000000, 2.165063509461101265 ) ) ;
#87814=DIRECTION ( 'NONE',  ( -4.274815082592931898E-19, -0.9999939076577903929, -0.003490651415223739937 ) ) ;
#87815=DIRECTION ( 'NONE',  ( 0.000000000000000000, 0.000000000000000000, 1.000000000000000000 ) ) ;
#87816=EDGE_LOOP ( 'NONE', ( #65312, #12630 ) ) ;
#87817=CARTESIAN_POINT ( 'NONE',  ( 0.8499999999999553468, 2.500000000000000000, -2.165063509461101710 ) ) ;
#87818=DIRECTION ( 'NONE',  ( 0.000000000000000000, -0.000000000000000000, 1.000000000000000000 ) ) ;
#87819=ADVANCED_FACE ( 'NONE', ( #55450 ), #16831, .T. ) ;
#87820=DIRECTION ( 'NONE',  ( 0.000000000000000000, -0.9999939076577903929, 0.003490651415223739937 ) ) ;
#87821=CARTESIAN_POINT ( 'NONE',  ( -0.8500000000000382805, 12.50000000000000000, -7.188010851410854052 ) ) ;
#87822=EDGE_CURVE ( 'NONE', #35339, #10073, #27266, .T. ) ;
#87823=DIRECTION ( 'NONE',  ( 0.000000000000000000, 1.000000000000000000, 0.000000000000000000 ) ) ;
#87824=VERTEX_POINT ( 'NONE', #128059 ) ;
#87825=ORIENTED_EDGE ( 'NONE', *, *, #88281, .T. ) ;
#87826=EDGE_CURVE ( 'NONE', #101170, #59036, #220, .T. ) ;
#87827=CIRCLE ( 'NONE', #31417, 0.06509327318403743123 ) ;
#87828=EDGE_CURVE ( 'NONE', #117628, #80777, #37799, .T. ) ;
#87829=FACE_OUTER_BOUND ( 'NONE', #14569, .T. ) ;
#87830=VECTOR ( 'NONE', #116277, 1000.000000000000000 ) ;
#87831=EDGE_CURVE ( 'NONE', #78070, #74183, #67097, .T. ) ;
#87832=ORIENTED_EDGE ( 'NONE', *, *, #87112, .F. ) ;
#87833=DIRECTION ( 'NONE',  ( -0.000000000000000000, -1.000000000000000000, -0.000000000000000000 ) ) ;
#87834=FACE_OUTER_BOUND ( 'NONE', #63510, .T. ) ;
#87836=CIRCLE ( 'NONE', #8418, 0.1000000000000002554 ) ;
#87837=EDGE_CURVE ( 'NONE', #49637, #69423, #23213, .T. ) ;
#87838=ORIENTED_EDGE ( 'NONE', *, *, #15453, .T. ) ;
#87840=CARTESIAN_POINT ( 'NONE',  ( 9.149999999999920419, 12.50000000000000000, 2.922977105672686982 ) ) ;
#87841=EDGE_CURVE ( 'NONE', #116200, #76636, #39953, .T. ) ;
#87842=CARTESIAN_POINT ( 'NONE',  ( -15.39999999999997904, 12.50000000000000000, 0.000000000000000000 ) ) ;
#87843=CARTESIAN_POINT ( 'NONE',  ( -6.050000000000020250, 12.50000000000000000, -6.841600689897078702 ) ) ;
#87844=ORIENTED_EDGE ( 'NONE', *, *, #78238, .T. ) ;
#87845=EDGE_CURVE ( 'NONE', #59380, #37927, #98419, .T. ) ;
#87846=DIRECTION ( 'NONE',  ( 0.000000000000000000, -0.000000000000000000, 1.000000000000000000 ) ) ;
#87847=DIRECTION ( 'NONE',  ( 0.000000000000000000, 0.000000000000000000, 1.000000000000000000 ) ) ;
#87848=EDGE_LOOP ( 'NONE', ( #53061, #116412, #111910, #32092 ) ) ;
#87849=CARTESIAN_POINT ( 'NONE',  ( 2.899999999999946620, 2.500000000000000000, -0.6928203230275542523 ) ) ;
#87850=DIRECTION ( 'NONE',  ( -0.000000000000000000, 1.000000000000000000, -0.000000000000000000 ) ) ;
#87851=CARTESIAN_POINT ( 'NONE',  ( 11.89999999999990798, 2.500000000000000000, -4.676537180435977881 ) ) ;
#87852=ORIENTED_EDGE ( 'NONE', *, *, #104492, .T. ) ;
#87853=CARTESIAN_POINT ( 'NONE',  ( 4.999999999999933387, 12.50000000000000000, 5.022947341949748790 ) ) ;
#87854=VERTEX_POINT ( 'NONE', #37747 ) ;
#87855=DIRECTION ( 'NONE',  ( 0.000000000000000000, 0.000000000000000000, -1.000000000000000000 ) ) ;
#87856=DIRECTION ( 'NONE',  ( 0.000000000000000000, 1.000000000000000000, 0.000000000000000000 ) ) ;
#87857=DIRECTION ( 'NONE',  ( -0.000000000000000000, -1.000000000000000000, -0.000000000000000000 ) ) ;
#87858=EDGE_LOOP ( 'NONE', ( #32826, #14962, #109191, #117251 ) ) ;
#87859=DIRECTION ( 'NONE',  ( 0.000000000000000000, 0.000000000000000000, -1.000000000000000000 ) ) ;
#87860=CONICAL_SURFACE ( 'NONE', #12650, 0.09999999999999982514, 0.003490658503988666988 ) ;
#87861=CARTESIAN_POINT ( 'NONE',  ( 0.1999999999999562961, 2.500000000000000000, 4.676537180435972552 ) ) ;
#87862=VERTEX_POINT ( 'NONE', #96635 ) ;
#87863=DIRECTION ( 'NONE',  ( -0.000000000000000000, 1.000000000000000000, -0.000000000000000000 ) ) ;
#87864=VERTEX_POINT ( 'NONE', #46937 ) ;
#87865=CONICAL_SURFACE ( 'NONE', #54430, 0.1000000000000002554, 0.003490658503988666988 ) ;
#87866=DIRECTION ( 'NONE',  ( 0.000000000000000000, 0.000000000000000000, 1.000000000000000000 ) ) ;
#87867=ADVANCED_FACE ( 'NONE', ( #107109 ), #16921, .T. ) ;
#87868=ORIENTED_EDGE ( 'NONE', *, *, #120752, .F. ) ;
#87869=DIRECTION ( 'NONE',  ( 0.000000000000000000, -0.000000000000000000, 1.000000000000000000 ) ) ;
#87870=DIRECTION ( 'NONE',  ( 0.000000000000000000, 0.000000000000000000, 1.000000000000000000 ) ) ;
#87871=EDGE_CURVE ( 'NONE', #47911, #27024, #35744, .T. ) ;
#87872=VERTEX_POINT ( 'NONE', #127416 ) ;
#87873=EDGE_LOOP ( 'NONE', ( #92413, #567, #90140, #95068 ) ) ;
#87874=CARTESIAN_POINT ( 'NONE',  ( 5.599999999999934808, 2.500000000000000000, -4.676537180435978769 ) ) ;
#87875=DIRECTION ( 'NONE',  ( 0.000000000000000000, 0.000000000000000000, 1.000000000000000000 ) ) ;
#87876=ORIENTED_EDGE ( 'NONE', *, *, #812, .F. ) ;
#87877=CIRCLE ( 'NONE', #79502, 0.06509327318403745899 ) ;
#87878=FACE_OUTER_BOUND ( 'NONE', #112170, .T. ) ;
#87879=DIRECTION ( 'NONE',  ( 0.000000000000000000, 0.000000000000000000, -1.000000000000000000 ) ) ;
#87880=AXIS2_PLACEMENT_3D ( 'NONE', #5749, #84973, #96086 ) ;
#87881=DIRECTION ( 'NONE',  ( 0.000000000000000000, 0.000000000000000000, 1.000000000000000000 ) ) ;
#87882=DIRECTION ( 'NONE',  ( 0.000000000000000000, 0.000000000000000000, 1.000000000000000000 ) ) ;
#87884=DIRECTION ( 'NONE',  ( -0.000000000000000000, 1.000000000000000000, -0.000000000000000000 ) ) ;
#87885=CIRCLE ( 'NONE', #71179, 0.06509327318403745899 ) ;
#87886=VERTEX_POINT ( 'NONE', #71070 ) ;
#87887=VERTEX_POINT ( 'NONE', #61258 ) ;
#87888=ORIENTED_EDGE ( 'NONE', *, *, #10373, .F. ) ;
#87889=ORIENTED_EDGE ( 'NONE', *, *, #64689, .T. ) ;
#87890=AXIS2_PLACEMENT_3D ( 'NONE', #107043, #47502, #17364 ) ;
#87891=LINE ( 'NONE', #19147, #110171 ) ;
#87892=CARTESIAN_POINT ( 'NONE',  ( -6.650000000000018119, 2.500000000000000000, -2.065063509461102065 ) ) ;
#87893=FACE_OUTER_BOUND ( 'NONE', #97218, .T. ) ;
#87894=EDGE_LOOP ( 'NONE', ( #47636, #96519, #110506, #58427 ) ) ;
#87895=FACE_BOUND ( 'NONE', #95982, .T. ) ;
#87896=ORIENTED_EDGE ( 'NONE', *, *, #99973, .T. ) ;
#87897=CARTESIAN_POINT ( 'NONE',  ( 6.699999999999930012, 12.50000000000000000, -4.330127018922201643 ) ) ;
#87898=CARTESIAN_POINT ( 'NONE',  ( 6.899999999999926636, 2.500000000000000000, -0.3464101615137782364 ) ) ;
#87899=FACE_OUTER_BOUND ( 'NONE', #48552, .T. ) ;
#87900=DIRECTION ( 'NONE',  ( 0.000000000000000000, 0.000000000000000000, 1.000000000000000000 ) ) ;
#87901=DIRECTION ( 'NONE',  ( -0.000000000000000000, 1.000000000000000000, -0.000000000000000000 ) ) ;
#87902=CARTESIAN_POINT ( 'NONE',  ( 9.599999999999914380, 2.500000000000000000, 4.230127018922196669 ) ) ;
#87903=EDGE_LOOP ( 'NONE', ( #56060, #67382 ) ) ;
#87904=CARTESIAN_POINT ( 'NONE',  ( -12.89999999999999147, 12.50000000000000000, 4.265033745738159077 ) ) ;
#87905=CARTESIAN_POINT ( 'NONE',  ( 4.199999999999939782, 2.500000000000000000, 0.09999999999999772959 ) ) ;
#87906=FACE_OUTER_BOUND ( 'NONE', #71032, .T. ) ;
#87907=ADVANCED_FACE ( 'NONE', ( #371 ), #104682, .T. ) ;
#87908=ORIENTED_EDGE ( 'NONE', *, *, #36147, .T. ) ;
#87909=ORIENTED_EDGE ( 'NONE', *, *, #47485, .T. ) ;
#87910=ORIENTED_EDGE ( 'NONE', *, *, #5794, .T. ) ;
#87911=EDGE_LOOP ( 'NONE', ( #60163, #85222, #23897, #33037 ) ) ;
#87912=CARTESIAN_POINT ( 'NONE',  ( 16.96615051717151701, -1.026750547570780547, -5.590381354654383017 ) ) ;
#87913=VECTOR ( 'NONE', #65741, 1000.000000000000000 ) ;
#87914=CARTESIAN_POINT ( 'NONE',  ( 4.149999999999941735, 12.50000000000000000, -1.472243186433550122 ) ) ;
#87915=VECTOR ( 'NONE', #88087, 1000.000000000000000 ) ;
#87916=ORIENTED_EDGE ( 'NONE', *, *, #41582, .F. ) ;
#87917=ORIENTED_EDGE ( 'NONE', *, *, #114046, .T. ) ;
#87918=VERTEX_POINT ( 'NONE', #120812 ) ;
#87919=DIRECTION ( 'NONE',  ( 0.000000000000000000, 0.000000000000000000, -1.000000000000000000 ) ) ;
#87920=EDGE_CURVE ( 'NONE', #89608, #49421, #14773, .T. ) ;
#87921=DIRECTION ( 'NONE',  ( 0.000000000000000000, 1.000000000000000000, 0.000000000000000000 ) ) ;
#87922=CARTESIAN_POINT ( 'NONE',  ( -5.600000000000020073, 2.500000000000000000, 0.2464101615137736789 ) ) ;
#87923=FACE_OUTER_BOUND ( 'NONE', #84165, .T. ) ;
#87924=DIRECTION ( 'NONE',  ( 0.000000000000000000, 0.000000000000000000, -1.000000000000000000 ) ) ;
#87925=CARTESIAN_POINT ( 'NONE',  ( 1.249999999999952482, 2.500000000000000000, -5.802370205355749988 ) ) ;
#87926=CIRCLE ( 'NONE', #104653, 0.09999999999999982514 ) ;
#87927=EDGE_CURVE ( 'NONE', #126243, #1900, #87948, .T. ) ;
#87928=CARTESIAN_POINT ( 'NONE',  ( 8.099999999999921485, 12.50000000000000000, -0.3464101615137783474 ) ) ;
#87929=EDGE_CURVE ( 'NONE', #39515, #49457, #29858, .T. ) ;
#87930=ORIENTED_EDGE ( 'NONE', *, *, #72533, .T. ) ;
#87931=DIRECTION ( 'NONE',  ( 0.000000000000000000, 0.000000000000000000, -1.000000000000000000 ) ) ;
#87932=ORIENTED_EDGE ( 'NONE', *, *, #103478, .T. ) ;
#87933=EDGE_LOOP ( 'NONE', ( #79042, #99186 ) ) ;
#87934=ORIENTED_EDGE ( 'NONE', *, *, #79108, .F. ) ;
#87935=EDGE_CURVE ( 'NONE', #87786, #118224, #4408, .T. ) ;
#87936=FACE_OUTER_BOUND ( 'NONE', #62019, .T. ) ;
#87937=ORIENTED_EDGE ( 'NONE', *, *, #109543, .F. ) ;
#87938=EDGE_CURVE ( 'NONE', #40642, #129526, #52458, .T. ) ;
#87939=ORIENTED_EDGE ( 'NONE', *, *, #64327, .T. ) ;
#87940=LINE ( 'NONE', #96472, #96643 ) ;
#87941=DIRECTION ( 'NONE',  ( 0.000000000000000000, 0.000000000000000000, 1.000000000000000000 ) ) ;
#87942=LINE ( 'NONE', #56557, #20673 ) ;
#87943=DIRECTION ( 'NONE',  ( -0.000000000000000000, -1.000000000000000000, -0.000000000000000000 ) ) ;
#87944=FACE_OUTER_BOUND ( 'NONE', #31582, .T. ) ;
#87945=VERTEX_POINT ( 'NONE', #20048 ) ;
#87946=CARTESIAN_POINT ( 'NONE',  ( -0.2000000000000408673, 2.500000000000000000, -3.983716857408426293 ) ) ;
#87947=CONICAL_SURFACE ( 'NONE', #110939, 0.09999999999999982514, 0.003490658503988666988 ) ;
#87948=CIRCLE ( 'NONE', #94229, 0.1000000000000000472 ) ;
#87950=CARTESIAN_POINT ( 'NONE',  ( -1.050000000000037792, 12.50000000000000000, 6.148780366869520009 ) ) ;
#87951=ORIENTED_EDGE ( 'NONE', *, *, #63810, .T. ) ;
#87953=DIRECTION ( 'NONE',  ( -0.000000000000000000, -1.000000000000000000, -0.000000000000000000 ) ) ;
#87954=EDGE_LOOP ( 'NONE', ( #3166, #42107 ) ) ;
#87955=LINE ( 'NONE', #99102, #105175 ) ;
#87956=CARTESIAN_POINT ( 'NONE',  ( 1.449999999999951772, 2.500000000000000000, -6.148780366869526226 ) ) ;
#87957=ORIENTED_EDGE ( 'NONE', *, *, #1690, .F. ) ;
#87958=AXIS2_PLACEMENT_3D ( 'NONE', #128119, #7026, #28635 ) ;
#87959=CIRCLE ( 'NONE', #37809, 0.06509327318403745899 ) ;
#87960=EDGE_CURVE ( 'NONE', #53806, #101537, #56645, .T. ) ;
#87961=DIRECTION ( 'NONE',  ( 0.000000000000000000, 0.000000000000000000, 1.000000000000000000 ) ) ;
#87962=ORIENTED_EDGE ( 'NONE', *, *, #107036, .F. ) ;
#87963=ORIENTED_EDGE ( 'NONE', *, *, #30771, .T. ) ;
#87964=CARTESIAN_POINT ( 'NONE',  ( -5.200000000000025935, 12.50000000000000000, -3.918623584224389056 ) ) ;
#87965=DIRECTION ( 'NONE',  ( -0.000000000000000000, -1.000000000000000000, -0.000000000000000000 ) ) ;
#87966=ADVANCED_FACE ( 'NONE', ( #99893 ), #115130, .T. ) ;
#87968=FACE_OUTER_BOUND ( 'NONE', #30503, .T. ) ;
#87969=EDGE_CURVE ( 'NONE', #127557, #103729, #110940, .T. ) ;
#87970=AXIS2_PLACEMENT_3D ( 'NONE', #83678, #32019, #82410 ) ;
#87971=CIRCLE ( 'NONE', #100508, 0.1000000000000002554 ) ;
#87972=DIRECTION ( 'NONE',  ( 0.000000000000000000, -0.000000000000000000, 1.000000000000000000 ) ) ;
#87973=DIRECTION ( 'NONE',  ( 0.000000000000000000, 1.000000000000000000, 0.000000000000000000 ) ) ;
#87974=EDGE_CURVE ( 'NONE', #117851, #110872, #127673, .T. ) ;
#87975=EDGE_CURVE ( 'NONE', #108330, #71667, #62930, .T. ) ;
#87976=ADVANCED_FACE ( 'NONE', ( #59342 ), #21159, .T. ) ;
#87977=CONICAL_SURFACE ( 'NONE', #33630, 0.09999999999999982514, 0.003490658503988666988 ) ;
#87979=VERTEX_POINT ( 'NONE', #129372 ) ;
#87980=DIRECTION ( 'NONE',  ( 0.000000000000000000, 0.000000000000000000, 1.000000000000000000 ) ) ;
#87981=CARTESIAN_POINT ( 'NONE',  ( 13.34999999999989662, 2.500000000000000000, -1.572243186433550211 ) ) ;
#87982=ORIENTED_EDGE ( 'NONE', *, *, #84271, .F. ) ;
#87983=ADVANCED_FACE ( 'NONE', ( #11503 ), #2278, .T. ) ;
#87984=DIRECTION ( 'NONE',  ( 0.000000000000000000, 1.000000000000000000, 0.000000000000000000 ) ) ;
#87985=LINE ( 'NONE', #36980, #115758 ) ;
#87986=CARTESIAN_POINT ( 'NONE',  ( -8.150000000000009237, 12.50000000000000000, 6.148780366869520009 ) ) ;
#87987=DIRECTION ( 'NONE',  ( 0.000000000000000000, 0.000000000000000000, 1.000000000000000000 ) ) ;
#87988=CARTESIAN_POINT ( 'NONE',  ( 14.34999999999989662, 2.500000000000000000, 1.918653347947321564 ) ) ;
#87989=ORIENTED_EDGE ( 'NONE', *, *, #63688, .T. ) ;
#87990=EDGE_CURVE ( 'NONE', #110679, #55365, #64974, .T. ) ;
#87991=ADVANCED_FACE ( 'NONE', ( #60623 ), #81634, .T. ) ;
#87992=FACE_OUTER_BOUND ( 'NONE', #56399, .T. ) ;
#87994=ORIENTED_EDGE ( 'NONE', *, *, #18216, .F. ) ;
#87995=FACE_OUTER_BOUND ( 'NONE', #129485, .T. ) ;
#87996=ORIENTED_EDGE ( 'NONE', *, *, #125569, .T. ) ;
#87997=ORIENTED_EDGE ( 'NONE', *, *, #59596, .T. ) ;
#87998=FACE_OUTER_BOUND ( 'NONE', #39487, .T. ) ;
#87999=AXIS2_PLACEMENT_3D ( 'NONE', #38904, #87943, #78814 ) ;
#88000=EDGE_LOOP ( 'NONE', ( #42999, #54419, #56933, #35723 ) ) ;
#88002=DIRECTION ( 'NONE',  ( 0.000000000000000000, 1.000000000000000000, 0.000000000000000000 ) ) ;
#88003=CARTESIAN_POINT ( 'NONE',  ( -15.79999999999998117, 12.50000000000000000, 0.06509327318403743123 ) ) ;
#88004=ORIENTED_EDGE ( 'NONE', *, *, #85274, .F. ) ;
#88005=DIRECTION ( 'NONE',  ( -0.000000000000000000, 1.000000000000000000, -0.000000000000000000 ) ) ;
#88006=DIRECTION ( 'NONE',  ( 0.000000000000000000, 0.000000000000000000, -1.000000000000000000 ) ) ;
#88007=ORIENTED_EDGE ( 'NONE', *, *, #97448, .T. ) ;
#88008=CIRCLE ( 'NONE', #119413, 0.06509327318403745899 ) ;
#88009=PLANE ( 'NONE',  #10951 ) ;
#88010=LINE ( 'NONE', #88686, #4882 ) ;
#88011=ORIENTED_EDGE ( 'NONE', *, *, #13563, .T. ) ;
#88012=ADVANCED_FACE ( 'NONE', ( #53371 ), #25253, .T. ) ;
#88013=VERTEX_POINT ( 'NONE', #93931 ) ;
#88014=ORIENTED_EDGE ( 'NONE', *, *, #115763, .T. ) ;
#88015=CARTESIAN_POINT ( 'NONE',  ( -11.44999999999999929, 2.500000000000000000, -6.248780366869523206 ) ) ;
#88016=LINE ( 'NONE', #78242, #125281 ) ;
#88017=LINE ( 'NONE', #58599, #111148 ) ;
#88018=FACE_BOUND ( 'NONE', #12691, .T. ) ;
#88019=ORIENTED_EDGE ( 'NONE', *, *, #102173, .F. ) ;
#88020=CARTESIAN_POINT ( 'NONE',  ( 12.89999999999990266, 12.50000000000000000, 3.702399969078682407 ) ) ;
#88021=DIRECTION ( 'NONE',  ( 0.000000000000000000, 0.000000000000000000, 1.000000000000000000 ) ) ;
#88022=EDGE_LOOP ( 'NONE', ( #84199, #123978 ) ) ;
#88023=EDGE_CURVE ( 'NONE', #84019, #54932, #32468, .T. ) ;
#88024=CARTESIAN_POINT ( 'NONE',  ( 10.84999999999991260, 12.50000000000000000, -1.407149913249512663 ) ) ;
#88025=AXIS2_PLACEMENT_3D ( 'NONE', #116417, #7106, #47706 ) ;
#88026=DIRECTION ( 'NONE',  ( 0.000000000000000000, -0.9999939076577903929, 0.003490651415223739937 ) ) ;
#88027=CARTESIAN_POINT ( 'NONE',  ( -11.25000000000000000, 12.50000000000000000, -7.188010851410850499 ) ) ;
#88028=CARTESIAN_POINT ( 'NONE',  ( 12.49999999999990230, 12.50000000000000000, -0.7579135962115916003 ) ) ;
#88029=DIRECTION ( 'NONE',  ( 0.000000000000000000, 1.000000000000000000, 0.000000000000000000 ) ) ;
#88030=CARTESIAN_POINT ( 'NONE',  ( 4.999999999999936939, 2.500000000000000000, -3.537306695894649966 ) ) ;
#88031=CIRCLE ( 'NONE', #94308, 0.1000000000000002554 ) ;
#88032=CIRCLE ( 'NONE', #44231, 0.1000000000000002554 ) ;
#88033=ORIENTED_EDGE ( 'NONE', *, *, #9581, .F. ) ;
#88034=ORIENTED_EDGE ( 'NONE', *, *, #88239, .F. ) ;
#88035=VERTEX_POINT ( 'NONE', #23242 ) ;
#88036=ORIENTED_EDGE ( 'NONE', *, *, #17581, .T. ) ;
#88037=ORIENTED_EDGE ( 'NONE', *, *, #30070, .F. ) ;
#88038=DIRECTION ( 'NONE',  ( 0.000000000000000000, 0.000000000000000000, 1.000000000000000000 ) ) ;
#88039=CARTESIAN_POINT ( 'NONE',  ( -9.400000000000007461, 2.500000000000000000, -0.4464101615137783252 ) ) ;
#88040=ORIENTED_EDGE ( 'NONE', *, *, #55924, .T. ) ;
#88041=FACE_BOUND ( 'NONE', #13714, .T. ) ;
#88042=DIRECTION ( 'NONE',  ( 0.000000000000000000, 0.000000000000000000, -1.000000000000000000 ) ) ;
#88043=CIRCLE ( 'NONE', #2363, 0.06509327318403745899 ) ;
#88044=CARTESIAN_POINT ( 'NONE',  ( 13.14999999999990088, 2.500000000000000000, 1.818653347947321475 ) ) ;
#88045=CARTESIAN_POINT ( 'NONE',  ( 13.74999999999989519, 2.500000000000000000, -2.857883832488653741 ) ) ;
#88046=DIRECTION ( 'NONE',  ( -0.000000000000000000, 1.000000000000000000, -0.000000000000000000 ) ) ;
#88047=DIRECTION ( 'NONE',  ( 0.000000000000000000, 0.000000000000000000, 1.000000000000000000 ) ) ;
#88048=VERTEX_POINT ( 'NONE', #112291 ) ;
#88049=DIRECTION ( 'NONE',  ( 0.000000000000000000, 0.000000000000000000, 1.000000000000000000 ) ) ;
#88050=AXIS2_PLACEMENT_3D ( 'NONE', #94134, #84314, #115046 ) ;
#88051=EDGE_LOOP ( 'NONE', ( #88864, #51538, #49310, #16250 ) ) ;
#88052=CIRCLE ( 'NONE', #79676, 0.1000000000000002554 ) ;
#88053=VERTEX_POINT ( 'NONE', #123383 ) ;
#88054=ORIENTED_EDGE ( 'NONE', *, *, #114602, .F. ) ;
#88055=AXIS2_PLACEMENT_3D ( 'NONE', #7660, #58080, #10258 ) ;
#88056=DIRECTION ( 'NONE',  ( 0.000000000000000000, 0.000000000000000000, 1.000000000000000000 ) ) ;
#88057=CARTESIAN_POINT ( 'NONE',  ( -0.8500000000000386136, 12.50000000000000000, 5.737276932171707422 ) ) ;
#88058=DIRECTION ( 'NONE',  ( -0.000000000000000000, 1.000000000000000000, -0.000000000000000000 ) ) ;
#88059=ORIENTED_EDGE ( 'NONE', *, *, #33874, .T. ) ;
#88060=DIRECTION ( 'NONE',  ( 0.000000000000000000, 0.000000000000000000, 1.000000000000000000 ) ) ;
#88061=AXIS2_PLACEMENT_3D ( 'NONE', #41699, #72437, #111711 ) ;
#88062=EDGE_CURVE ( 'NONE', #112816, #21177, #18995, .T. ) ;
#88063=CARTESIAN_POINT ( 'NONE',  ( -12.89999999999999147, 2.500000000000000000, -4.330127018922198978 ) ) ;
#88064=CARTESIAN_POINT ( 'NONE',  ( -11.44999999999999929, 12.50000000000000000, -6.148780366869522673 ) ) ;
#88065=AXIS2_PLACEMENT_3D ( 'NONE', #20462, #18518, #58464 ) ;
#88066=CIRCLE ( 'NONE', #8651, 0.1000000000000000056 ) ;
#88068=DIRECTION ( 'NONE',  ( 0.000000000000000000, 0.000000000000000000, -1.000000000000000000 ) ) ;
#88069=DIRECTION ( 'NONE',  ( 0.000000000000000000, 1.000000000000000000, 0.000000000000000000 ) ) ;
#88070=ADVANCED_FACE ( 'NONE', ( #71710 ), #69172, .T. ) ;
#88071=DIRECTION ( 'NONE',  ( -0.000000000000000000, 1.000000000000000000, -0.000000000000000000 ) ) ;
#88072=ADVANCED_FACE ( 'NONE', ( #113572 ), #43559, .T. ) ;
#88073=ORIENTED_EDGE ( 'NONE', *, *, #22512, .T. ) ;
#88074=CARTESIAN_POINT ( 'NONE',  ( -9.400000000000009237, 12.50000000000000000, -4.611443907251936203 ) ) ;
#88075=EDGE_LOOP ( 'NONE', ( #38453, #23093, #5732, #38538 ) ) ;
#88076=EDGE_LOOP ( 'NONE', ( #8769, #90342, #73144, #123599 ) ) ;
#88077=DIRECTION ( 'NONE',  ( 0.000000000000000000, 0.000000000000000000, 1.000000000000000000 ) ) ;
#88078=ADVANCED_FACE ( 'NONE', ( #82841 ), #46200, .T. ) ;
#88079=CARTESIAN_POINT ( 'NONE',  ( -7.700000000000014388, 12.50000000000000000, -0.3464101615137782364 ) ) ;
#88080=DIRECTION ( 'NONE',  ( 0.000000000000000000, 0.000000000000000000, 1.000000000000000000 ) ) ;
#88082=ORIENTED_EDGE ( 'NONE', *, *, #32122, .F. ) ;
#88083=VERTEX_POINT ( 'NONE', #124687 ) ;
#88085=CARTESIAN_POINT ( 'NONE',  ( -5.850000000000021849, 12.50000000000000000, -2.857883832488653741 ) ) ;
#88087=DIRECTION ( 'NONE',  ( -4.274815082592931898E-19, -0.9999939076577903929, -0.003490651415223739937 ) ) ;
#88088=ORIENTED_EDGE ( 'NONE', *, *, #30240, .T. ) ;
#88089=ORIENTED_EDGE ( 'NONE', *, *, #37034, .F. ) ;
#88090=VECTOR ( 'NONE', #60646, 1000.000000000000000 ) ;
#88091=AXIS2_PLACEMENT_3D ( 'NONE', #33572, #63020, #113405 ) ;
#88092=PLANE ( 'NONE',  #66990 ) ;
#88093=ORIENTED_EDGE ( 'NONE', *, *, #94823, .F. ) ;
#88094=DIRECTION ( 'NONE',  ( -0.000000000000000000, 1.000000000000000000, -0.000000000000000000 ) ) ;
#88095=CONICAL_SURFACE ( 'NONE', #104835, 0.09999999999999982514, 0.003490658503988666988 ) ;
#88096=CARTESIAN_POINT ( 'NONE',  ( -6.249999999999981348, 2.500000000000000000, 2.165063509461097713 ) ) ;
#88097=ORIENTED_EDGE ( 'NONE', *, *, #63257, .T. ) ;
#88098=PLANE ( 'NONE',  #69091 ) ;
#88099=VECTOR ( 'NONE', #47545, 1000.000000000000000 ) ;
#88100=PLANE ( 'NONE',  #98539 ) ;
#88101=DIRECTION ( 'NONE',  ( 0.000000000000000000, 1.000000000000000000, 0.000000000000000000 ) ) ;
#88102=CONICAL_SURFACE ( 'NONE', #31703, 0.09999999999999982514, 0.003490658503988666988 ) ;
#88103=DIRECTION ( 'NONE',  ( 0.000000000000000000, 1.000000000000000000, 0.000000000000000000 ) ) ;
#88104=EDGE_LOOP ( 'NONE', ( #65836, #43324 ) ) ;
#88105=CONICAL_SURFACE ( 'NONE', #46358, 0.09999999999999999167, 0.003490658503988666988 ) ;
#88106=CARTESIAN_POINT ( 'NONE',  ( 6.049999999999932321, 2.500000000000000000, 1.818653347947321475 ) ) ;
#88107=ORIENTED_EDGE ( 'NONE', *, *, #55461, .F. ) ;
#88108=ORIENTED_EDGE ( 'NONE', *, *, #23123, .F. ) ;
#88109=DIRECTION ( 'NONE',  ( 0.000000000000000000, 0.000000000000000000, -1.000000000000000000 ) ) ;
#88110=CARTESIAN_POINT ( 'NONE',  ( -7.050000000000013145, 12.50000000000000000, 6.495190528383297135 ) ) ;
#88111=CARTESIAN_POINT ( 'NONE',  ( 13.14999999999990088, 12.50000000000000000, 1.818653347947321475 ) ) ;
#88112=CARTESIAN_POINT ( 'NONE',  ( -9.350000000000006750, 2.500000000000000000, -1.818653347947325916 ) ) ;
#88113=DIRECTION ( 'NONE',  ( 0.000000000000000000, 0.000000000000000000, 1.000000000000000000 ) ) ;
#88114=CARTESIAN_POINT ( 'NONE',  ( 14.99999999999989164, 12.50000000000000000, 0.6277270498435120194 ) ) ;
#88115=FACE_OUTER_BOUND ( 'NONE', #68728, .T. ) ;
#88116=CARTESIAN_POINT ( 'NONE',  ( -8.749999999999976907, 2.500000000000000000, -6.495190528383297135 ) ) ;
#88117=FACE_OUTER_BOUND ( 'NONE', #93052, .T. ) ;
#88118=EDGE_CURVE ( 'NONE', #69422, #109159, #79651, .T. ) ;
#88119=EDGE_CURVE ( 'NONE', #107424, #39659, #21248, .T. ) ;
#88120=EDGE_CURVE ( 'NONE', #125152, #92801, #54599, .T. ) ;
#88121=CARTESIAN_POINT ( 'NONE',  ( 9.599999999999917932, 2.500000000000000000, -0.6928203230275541413 ) ) ;
#88122=AXIS2_PLACEMENT_3D ( 'NONE', #103303, #5719, #92844 ) ;
#88123=CONICAL_SURFACE ( 'NONE', #113281, 0.1000000000000002554, 0.003490658503988666988 ) ;
#88124=VERTEX_POINT ( 'NONE', #65091 ) ;
#88125=EDGE_CURVE ( 'NONE', #64242, #97332, #73476, .T. ) ;
#88126=CARTESIAN_POINT ( 'NONE',  ( 5.849999999999931255, 2.500000000000000000, 2.857883832488649301 ) ) ;
#88127=CARTESIAN_POINT ( 'NONE',  ( 8.349999999999919709, 2.500000000000000000, -1.572243186433550211 ) ) ;
#88128=CARTESIAN_POINT ( 'NONE',  ( 12.94999999999990337, 2.500000000000000000, 2.065063509461097624 ) ) ;
#88129=DIRECTION ( 'NONE',  ( 0.000000000000000000, 1.000000000000000000, 0.000000000000000000 ) ) ;
#88130=FACE_OUTER_BOUND ( 'NONE', #26211, .T. ) ;
#88131=CIRCLE ( 'NONE', #6551, 0.06509327318403745899 ) ;
#88132=VECTOR ( 'NONE', #22621, 1000.000000000000000 ) ;
#88133=ORIENTED_EDGE ( 'NONE', *, *, #33585, .F. ) ;
#88134=EDGE_CURVE ( 'NONE', #74283, #22803, #19083, .T. ) ;
#88135=CARTESIAN_POINT ( 'NONE',  ( 10.19999999999991225, 2.500000000000000000, -4.576537180435978236 ) ) ;
#88136=AXIS2_PLACEMENT_3D ( 'NONE', #101413, #83066, #122985 ) ;
#88138=AXIS2_PLACEMENT_3D ( 'NONE', #99921, #400, #30555 ) ;
#88140=CARTESIAN_POINT ( 'NONE',  ( -1.650000000000034772, 2.500000000000000000, 2.165063509461097713 ) ) ;
#88141=EDGE_LOOP ( 'NONE', ( #76585, #103619, #114009, #43849 ) ) ;
#88142=EDGE_CURVE ( 'NONE', #115638, #97971, #37979, .T. ) ;
#88143=VECTOR ( 'NONE', #122802, 1000.000000000000000 ) ;
#88144=EDGE_LOOP ( 'NONE', ( #118678, #124938, #83340, #108050 ) ) ;
#88147=VERTEX_POINT ( 'NONE', #46117 ) ;
#88148=ORIENTED_EDGE ( 'NONE', *, *, #48253, .F. ) ;
#88149=CIRCLE ( 'NONE', #31759, 0.1000000000000000472 ) ;
#88150=ORIENTED_EDGE ( 'NONE', *, *, #120422, .T. ) ;
#88151=AXIS2_PLACEMENT_3D ( 'NONE', #43041, #13537, #63942 ) ;
#88152=CARTESIAN_POINT ( 'NONE',  ( 13.74999999999989875, 12.50000000000000000, 1.472243186433545459 ) ) ;
#88153=CIRCLE ( 'NONE', #121626, 0.09999999999999982514 ) ;
#88154=DIRECTION ( 'NONE',  ( 0.000000000000000000, 0.000000000000000000, 1.000000000000000000 ) ) ;
#88155=DIRECTION ( 'NONE',  ( 0.000000000000000000, 0.000000000000000000, 1.000000000000000000 ) ) ;
#88156=CARTESIAN_POINT ( 'NONE',  ( 4.599999999999937472, 2.500000000000000000, 0.6928203230275494784 ) ) ;
#88157=ORIENTED_EDGE ( 'NONE', *, *, #124397, .F. ) ;
#88158=AXIS2_PLACEMENT_3D ( 'NONE', #125719, #65526, #105464 ) ;
#88159=FACE_OUTER_BOUND ( 'NONE', #96266, .T. ) ;
#88160=ORIENTED_EDGE ( 'NONE', *, *, #13821, .T. ) ;
#88161=CARTESIAN_POINT ( 'NONE',  ( 14.39999999999989555, 2.500000000000000000, 0.3464101615137736845 ) ) ;
#88162=CARTESIAN_POINT ( 'NONE',  ( 16.04820284965659027, -1.499999999999968026, -6.585610464672694064 ) ) ;
#88163=CARTESIAN_POINT ( 'NONE',  ( 17.33812564108900389, 2.538896947917175684, 5.379288978442783531 ) ) ;
#88164=CARTESIAN_POINT ( 'NONE',  ( -1.650000000000034328, 2.500000000000000000, -7.188010851410854052 ) ) ;
#88165=CARTESIAN_POINT ( 'NONE',  ( 9.399999999999918643, 2.500000000000000000, -0.4464101615137782142 ) ) ;
#88166=VERTEX_POINT ( 'NONE', #46774 ) ;
#88169=ORIENTED_EDGE ( 'NONE', *, *, #93050, .F. ) ;
#88170=EDGE_LOOP ( 'NONE', ( #8884, #36467 ) ) ;
#88171=DIRECTION ( 'NONE',  ( 0.000000000000000000, -0.000000000000000000, 1.000000000000000000 ) ) ;
#88172=DIRECTION ( 'NONE',  ( 0.000000000000000000, 0.000000000000000000, 1.000000000000000000 ) ) ;
#88173=FACE_OUTER_BOUND ( 'NONE', #105389, .T. ) ;
#88174=FACE_BOUND ( 'NONE', #7486, .T. ) ;
#88175=DIRECTION ( 'NONE',  ( 0.000000000000000000, 1.000000000000000000, 0.000000000000000000 ) ) ;
#88176=DIRECTION ( 'NONE',  ( -0.000000000000000000, 1.000000000000000000, -0.000000000000000000 ) ) ;
#88177=CARTESIAN_POINT ( 'NONE',  ( 0.8499999999999536815, 12.50000000000000000, 6.495190528383297135 ) ) ;
#88178=CARTESIAN_POINT ( 'NONE',  ( 11.84999999999990727, 2.500000000000000000, -1.818653347947326138 ) ) ;
#88179=EDGE_CURVE ( 'NONE', #127460, #10341, #97154, .T. ) ;
#88180=CIRCLE ( 'NONE', #48503, 0.06509327318403745899 ) ;
#88181=CARTESIAN_POINT ( 'NONE',  ( -10.60000000000000142, 2.500000000000000000, -0.4464101615137782142 ) ) ;
#88182=CIRCLE ( 'NONE', #56887, 0.06509327318403745899 ) ;
#88184=DIRECTION ( 'NONE',  ( 0.000000000000000000, 0.000000000000000000, -1.000000000000000000 ) ) ;
#88185=AXIS2_PLACEMENT_3D ( 'NONE', #123923, #94461, #34289 ) ;
#88186=AXIS2_PLACEMENT_3D ( 'NONE', #37935, #77847, #7168 ) ;
#88187=DIRECTION ( 'NONE',  ( 0.000000000000000000, 0.000000000000000000, 1.000000000000000000 ) ) ;
#88188=ORIENTED_EDGE ( 'NONE', *, *, #56967, .F. ) ;
#88189=ORIENTED_EDGE ( 'NONE', *, *, #92894, .F. ) ;
#88190=ORIENTED_EDGE ( 'NONE', *, *, #29178, .F. ) ;
#88191=ORIENTED_EDGE ( 'NONE', *, *, #10807, .F. ) ;
#88192=CIRCLE ( 'NONE', #84004, 0.06509327318403745899 ) ;
#88193=AXIS2_PLACEMENT_3D ( 'NONE', #36841, #116028, #76759 ) ;
#88194=LINE ( 'NONE', #29314, #69484 ) ;
#88195=FACE_BOUND ( 'NONE', #20172, .T. ) ;
#88196=AXIS2_PLACEMENT_3D ( 'NONE', #67780, #59280, #37691 ) ;
#88197=CARTESIAN_POINT ( 'NONE',  ( 1.899999999999951283, 2.500000000000000000, -0.2464101615137782308 ) ) ;
#88198=VERTEX_POINT ( 'NONE', #37599 ) ;
#88199=DIRECTION ( 'NONE',  ( -0.000000000000000000, -1.000000000000000000, -0.000000000000000000 ) ) ;
#88200=DIRECTION ( 'NONE',  ( 0.000000000000000000, 0.000000000000000000, 1.000000000000000000 ) ) ;
#88201=DIRECTION ( 'NONE',  ( -0.000000000000000000, -1.000000000000000000, -0.000000000000000000 ) ) ;
#88202=DIRECTION ( 'NONE',  ( -0.000000000000000000, -1.000000000000000000, -0.000000000000000000 ) ) ;
#88203=ORIENTED_EDGE ( 'NONE', *, *, #87389, .T. ) ;
#88205=PLANE ( 'NONE',  #9487 ) ;
#88206=EDGE_LOOP ( 'NONE', ( #128320, #71202, #36049, #51998 ) ) ;
#88207=ORIENTED_EDGE ( 'NONE', *, *, #115752, .T. ) ;
#88208=DIRECTION ( 'NONE',  ( -0.000000000000000000, -1.000000000000000000, -0.000000000000000000 ) ) ;
#88209=DIRECTION ( 'NONE',  ( 0.000000000000000000, 1.000000000000000000, 0.000000000000000000 ) ) ;
#88210=ADVANCED_FACE ( 'NONE', ( #15345 ), #37890, .T. ) ;
#88211=ORIENTED_EDGE ( 'NONE', *, *, #16900, .F. ) ;
#88212=CONICAL_SURFACE ( 'NONE', #31819, 0.1000000000000002554, 0.003490658503988666988 ) ;
#88213=ADVANCED_FACE ( 'NONE', ( #116778 ), #117369, .T. ) ;
#88214=LINE ( 'NONE', #129492, #44665 ) ;
#88215=DIRECTION ( 'NONE',  ( 0.000000000000000000, -0.000000000000000000, 1.000000000000000000 ) ) ;
#88216=VERTEX_POINT ( 'NONE', #36320 ) ;
#88217=CARTESIAN_POINT ( 'NONE',  ( -5.200000000000020606, 12.50000000000000000, 3.983716857408420964 ) ) ;
#88218=ORIENTED_EDGE ( 'NONE', *, *, #85728, .T. ) ;
#88219=ADVANCED_FACE ( 'NONE', ( #17943 ), #57885, .T. ) ;
#88220=DIRECTION ( 'NONE',  ( -0.000000000000000000, 1.000000000000000000, -0.000000000000000000 ) ) ;
#88221=ADVANCED_FACE ( 'NONE', ( #74936 ), #111023, .T. ) ;
#88222=ORIENTED_EDGE ( 'NONE', *, *, #12712, .T. ) ;
#88223=DIRECTION ( 'NONE',  ( 0.000000000000000000, 1.000000000000000000, 0.000000000000000000 ) ) ;
#88224=CONICAL_SURFACE ( 'NONE', #79938, 0.1000000000000002554, 0.003490658503988666988 ) ;
#88225=FACE_BOUND ( 'NONE', #4157, .T. ) ;
#88226=CONICAL_SURFACE ( 'NONE', #23404, 0.09999999999999999167, 0.003490658503988666988 ) ;
#88227=ORIENTED_EDGE ( 'NONE', *, *, #81361, .T. ) ;
#88228=AXIS2_PLACEMENT_3D ( 'NONE', #15373, #26513, #87980 ) ;
#88230=ORIENTED_EDGE ( 'NONE', *, *, #114338, .T. ) ;
#88231=DIRECTION ( 'NONE',  ( -0.000000000000000000, -1.000000000000000000, -0.000000000000000000 ) ) ;
#88232=LINE ( 'NONE', #7758, #36182 ) ;
#88233=ADVANCED_FACE ( 'NONE', ( #116138 ), #100662, .T. ) ;
#88234=ADVANCED_FACE ( 'NONE', ( #26487 ), #71321, .T. ) ;
#88235=DIRECTION ( 'NONE',  ( 0.000000000000000000, 0.000000000000000000, -1.000000000000000000 ) ) ;
#88236=ADVANCED_FACE ( 'NONE', ( #75567 ), #31638, .T. ) ;
#88238=EDGE_CURVE ( 'NONE', #78195, #87945, #88032, .T. ) ;
#88239=EDGE_CURVE ( 'NONE', #89132, #105744, #23299, .T. ) ;
#88240=DIRECTION ( 'NONE',  ( 0.000000000000000000, 0.000000000000000000, -1.000000000000000000 ) ) ;
#88241=CONICAL_SURFACE ( 'NONE', #94519, 0.09999999999999982514, 0.003490658503988666988 ) ;
#88242=ORIENTED_EDGE ( 'NONE', *, *, #28281, .T. ) ;
#88243=EDGE_LOOP ( 'NONE', ( #44409, #64455 ) ) ;
#88246=DIRECTION ( 'NONE',  ( 0.000000000000000000, 0.000000000000000000, 1.000000000000000000 ) ) ;
#88247=LINE ( 'NONE', #100653, #13864 ) ;
#88248=CONICAL_SURFACE ( 'NONE', #115437, 0.09999999999999999167, 0.003490658503988666988 ) ;
#88249=FACE_OUTER_BOUND ( 'NONE', #92008, .T. ) ;
#88250=EDGE_LOOP ( 'NONE', ( #39330, #84213, #18309, #48642 ) ) ;
#88251=EDGE_LOOP ( 'NONE', ( #85746, #69812, #101833, #7405 ) ) ;
#88252=ORIENTED_EDGE ( 'NONE', *, *, #43777, .F. ) ;
#88253=EDGE_CURVE ( 'NONE', #32556, #10759, #108969, .T. ) ;
#88254=FACE_OUTER_BOUND ( 'NONE', #61865, .T. ) ;
#88255=CIRCLE ( 'NONE', #31849, 0.06509327318403745899 ) ;
#88256=FACE_OUTER_BOUND ( 'NONE', #97373, .T. ) ;
#88258=CARTESIAN_POINT ( 'NONE',  ( 9.149999999999918643, 2.500000000000000000, 2.065063509461097624 ) ) ;
#88259=AXIS2_PLACEMENT_3D ( 'NONE', #85009, #124946, #73910 ) ;
#88260=CARTESIAN_POINT ( 'NONE',  ( 13.14999999999990088, 12.50000000000000000, 2.511473670974873507 ) ) ;
#88261=CARTESIAN_POINT ( 'NONE',  ( -11.69999999999999574, 12.50000000000000000, 4.395220292106234439 ) ) ;
#88262=DIRECTION ( 'NONE',  ( 0.000000000000000000, 0.000000000000000000, 1.000000000000000000 ) ) ;
#88263=DIRECTION ( 'NONE',  ( 0.000000000000000000, 0.000000000000000000, 1.000000000000000000 ) ) ;
#88265=VERTEX_POINT ( 'NONE', #70278 ) ;
#88266=ORIENTED_EDGE ( 'NONE', *, *, #99350, .F. ) ;
#88267=CARTESIAN_POINT ( 'NONE',  ( -3.350000000000029399, 2.500000000000000000, 6.395190528383296602 ) ) ;
#88268=DIRECTION ( 'NONE',  ( -0.000000000000000000, 1.000000000000000000, -0.000000000000000000 ) ) ;
#88269=ORIENTED_EDGE ( 'NONE', *, *, #86142, .F. ) ;
#88270=ORIENTED_EDGE ( 'NONE', *, *, #8617, .T. ) ;
#88272=CARTESIAN_POINT ( 'NONE',  ( 7.049999999999926992, 2.500000000000000000, 2.165063509461097713 ) ) ;
#88273=CARTESIAN_POINT ( 'NONE',  ( 4.999999999999971578, 12.50000000000000000, -2.276824562219559311E-15 ) ) ;
#88274=DIRECTION ( 'NONE',  ( 0.000000000000000000, -0.9999939076577903929, 0.003490651415223739937 ) ) ;
#88275=DIRECTION ( 'NONE',  ( 0.000000000000000000, 0.000000000000000000, 1.000000000000000000 ) ) ;
#88276=AXIS2_PLACEMENT_3D ( 'NONE', #50710, #297, #89979 ) ;
#88277=CARTESIAN_POINT ( 'NONE',  ( -5.800000000000018474, 2.500000000000000000, 4.230127018922196669 ) ) ;
#88278=DIRECTION ( 'NONE',  ( -4.274815082592931898E-19, -0.9999939076577903929, -0.003490651415223739937 ) ) ;
#88279=AXIS2_PLACEMENT_3D ( 'NONE', #87849, #127787, #6065 ) ;
#88280=CIRCLE ( 'NONE', #11018, 0.06509327318403745899 ) ;
#88281=EDGE_CURVE ( 'NONE', #39517, #33308, #100377, .T. ) ;
#88282=EDGE_CURVE ( 'NONE', #52515, #52645, #99743, .T. ) ;
#88283=DIRECTION ( 'NONE',  ( 0.000000000000000000, 0.000000000000000000, 1.000000000000000000 ) ) ;
#88284=CIRCLE ( 'NONE', #119692, 0.09999999999999982514 ) ;
#88285=ORIENTED_EDGE ( 'NONE', *, *, #101355, .F. ) ;
#88286=CONICAL_SURFACE ( 'NONE', #69517, 0.1000000000000002554, 0.003490658503988666988 ) ;
#88287=ADVANCED_FACE ( 'NONE', ( #40835 ), #10051, .F. ) ;
#88288=CONICAL_SURFACE ( 'NONE', #71587, 0.09999999999999982514, 0.003490658503988666988 ) ;
#88289=EDGE_LOOP ( 'NONE', ( #67155, #74496 ) ) ;
#88290=AXIS2_PLACEMENT_3D ( 'NONE', #34351, #5494, #33689 ) ;
#88291=AXIS2_PLACEMENT_3D ( 'NONE', #60136, #97454, #8416 ) ;
#88292=VERTEX_POINT ( 'NONE', #886 ) ;
#88293=EDGE_CURVE ( 'NONE', #89801, #76324, #65061, .T. ) ;
#88294=ORIENTED_EDGE ( 'NONE', *, *, #24584, .F. ) ;
#88295=CARTESIAN_POINT ( 'NONE',  ( 11.24999999999994316, 12.50000000000000000, -6.430097255199264339 ) ) ;
#88296=DIRECTION ( 'NONE',  ( 0.000000000000000000, 0.000000000000000000, 1.000000000000000000 ) ) ;
#88297=AXIS2_PLACEMENT_3D ( 'NONE', #22167, #92162, #101997 ) ;
#88298=EDGE_CURVE ( 'NONE', #65655, #39561, #96457, .T. ) ;
#88299=ORIENTED_EDGE ( 'NONE', *, *, #75659, .F. ) ;
#88300=EDGE_CURVE ( 'NONE', #18873, #21324, #40048, .T. ) ;
#88301=CARTESIAN_POINT ( 'NONE',  ( -11.84999999999999787, 2.500000000000000000, -6.248780366869523206 ) ) ;
#88302=CARTESIAN_POINT ( 'NONE',  ( 17.50000000000000000, 0.9166666666666684060, -3.432456362931489036 ) ) ;
#88303=ADVANCED_FACE ( 'NONE', ( #19891 ), #10063, .T. ) ;
#88304=CARTESIAN_POINT ( 'NONE',  ( 4.199999999999941558, 2.500000000000000000, -4.230127018922201998 ) ) ;
#88305=FACE_OUTER_BOUND ( 'NONE', #69700, .T. ) ;
#88306=ORIENTED_EDGE ( 'NONE', *, *, #68210, .T. ) ;
#88307=CARTESIAN_POINT ( 'NONE',  ( 7.699999999999923794, 2.500000000000000000, -3.883716857408426648 ) ) ;
#88308=EDGE_CURVE ( 'NONE', #106514, #88607, #52557, .T. ) ;
#88309=AXIS2_PLACEMENT_3D ( 'NONE', #69167, #116342, #48918 ) ;
#88310=DIRECTION ( 'NONE',  ( 0.000000000000000000, -0.9999939076577903929, 0.003490651415223739937 ) ) ;
#88311=ORIENTED_EDGE ( 'NONE', *, *, #107055, .F. ) ;
#88312=EDGE_LOOP ( 'NONE', ( #55649, #112630, #102998, #18831 ) ) ;
#88313=ORIENTED_EDGE ( 'NONE', *, *, #44667, .F. ) ;
#88314=DIRECTION ( 'NONE',  ( 0.000000000000000000, 1.000000000000000000, 0.000000000000000000 ) ) ;
#88315=CONICAL_SURFACE ( 'NONE', #75804, 0.09999999999999982514, 0.003490658503988666988 ) ;
#88316=DIRECTION ( 'NONE',  ( 0.000000000000000000, 0.000000000000000000, 1.000000000000000000 ) ) ;
#88317=MECHANICAL_DESIGN_GEOMETRIC_PRESENTATION_REPRESENTATION('',(#10944),#36121);
#88318=ORIENTED_EDGE ( 'NONE', *, *, #21182, .F. ) ;
#88319=CARTESIAN_POINT ( 'NONE',  ( -10.45000000000000462, 12.50000000000000000, -6.560283801567336148 ) ) ;
#88320=DIRECTION ( 'NONE',  ( -0.000000000000000000, -1.000000000000000000, -0.000000000000000000 ) ) ;
#88322=DIRECTION ( 'NONE',  ( 0.000000000000000000, 0.000000000000000000, 1.000000000000000000 ) ) ;
#88323=ADVANCED_FACE ( 'NONE', ( #40176 ), #83938, .T. ) ;
#88324=CIRCLE ( 'NONE', #119638, 0.1000000000000002554 ) ;
#88325=ORIENTED_EDGE ( 'NONE', *, *, #118237, .F. ) ;
#88326=CARTESIAN_POINT ( 'NONE',  ( -12.89999999999999325, 12.50000000000000000, 0.6928203230275535862 ) ) ;
#88327=ORIENTED_EDGE ( 'NONE', *, *, #119805, .F. ) ;
#88328=ORIENTED_EDGE ( 'NONE', *, *, #102585, .T. ) ;
#88329=DIRECTION ( 'NONE',  ( -0.000000000000000000, 1.000000000000000000, -0.000000000000000000 ) ) ;
#88330=FACE_OUTER_BOUND ( 'NONE', #97621, .T. ) ;
#88331=FACE_BOUND ( 'NONE', #110558, .T. ) ;
#88332=CARTESIAN_POINT ( 'NONE',  ( -15.79999999999998117, 2.500000000000000000, 0.000000000000000000 ) ) ;
#88333=CIRCLE ( 'NONE', #46589, 0.1000000000000002554 ) ;
#88334=DIRECTION ( 'NONE',  ( -0.000000000000000000, 1.000000000000000000, -0.000000000000000000 ) ) ;
#88335=CIRCLE ( 'NONE', #100869, 0.09999999999999982514 ) ;
#88336=CARTESIAN_POINT ( 'NONE',  ( -12.89999999999999147, 12.50000000000000000, 4.330127018922196314 ) ) ;
#88337=ADVANCED_FACE ( 'NONE', ( #80095 ), #127902, .T. ) ;
#88338=AXIS2_PLACEMENT_3D ( 'NONE', #43871, #102758, #73300 ) ;
#88339=AXIS2_PLACEMENT_3D ( 'NONE', #122750, #128893, #103760 ) ;
#88340=AXIS2_PLACEMENT_3D ( 'NONE', #76519, #116419, #45775 ) ;
#88341=VERTEX_POINT ( 'NONE', #49365 ) ;
#88342=DIRECTION ( 'NONE',  ( 0.000000000000000000, 0.000000000000000000, 1.000000000000000000 ) ) ;
#88343=PLANE ( 'NONE',  #88699 ) ;
#88344=CARTESIAN_POINT ( 'NONE',  ( 15.59999999999988951, 2.500000000000000000, 0.3464101615137735735 ) ) ;
#88345=AXIS2_PLACEMENT_3D ( 'NONE', #97395, #47667, #86926 ) ;
#88346=DIRECTION ( 'NONE',  ( 0.000000000000000000, 0.000000000000000000, -1.000000000000000000 ) ) ;
#88347=VERTEX_POINT ( 'NONE', #38911 ) ;
#88348=FACE_OUTER_BOUND ( 'NONE', #101349, .T. ) ;
#88349=FACE_OUTER_BOUND ( 'NONE', #108603, .T. ) ;
#88350=CONICAL_SURFACE ( 'NONE', #84252, 0.09999999999999982514, 0.003490658503988666988 ) ;
#88351=ORIENTED_EDGE ( 'NONE', *, *, #118549, .F. ) ;
#88352=ORIENTED_EDGE ( 'NONE', *, *, #46155, .F. ) ;
#88353=DIRECTION ( 'NONE',  ( 0.000000000000000000, -0.000000000000000000, 1.000000000000000000 ) ) ;
#88354=EDGE_CURVE ( 'NONE', #24335, #97955, #113181, .T. ) ;
#88355=CARTESIAN_POINT ( 'NONE',  ( -6.650000000000014566, 2.500000000000000000, 1.472243186433545459 ) ) ;
#88356=FACE_BOUND ( 'NONE', #19939, .T. ) ;
#88357=CARTESIAN_POINT ( 'NONE',  ( -13.74999999999995381, 2.500000000000000000, -2.165063509461099489 ) ) ;
#88358=ORIENTED_EDGE ( 'NONE', *, *, #118446, .T. ) ;
#88359=DIRECTION ( 'NONE',  ( 0.000000000000000000, -0.000000000000000000, 1.000000000000000000 ) ) ;
#88360=VERTEX_POINT ( 'NONE', #119360 ) ;
#88361=AXIS2_PLACEMENT_3D ( 'NONE', #83149, #42586, #102135 ) ;
#88362=ORIENTED_EDGE ( 'NONE', *, *, #42204, .T. ) ;
#88363=CARTESIAN_POINT ( 'NONE',  ( 8.749999999999920064, 2.500000000000000000, 5.802370205355744659 ) ) ;
#88364=VECTOR ( 'NONE', #64164, 1000.000000000000000 ) ;
#88366=ORIENTED_EDGE ( 'NONE', *, *, #96390, .F. ) ;
#88367=DIRECTION ( 'NONE',  ( -4.274815082592931898E-19, -0.9999939076577903929, -0.003490651415223739937 ) ) ;
#88368=FACE_OUTER_BOUND ( 'NONE', #63014, .T. ) ;
#88370=AXIS2_PLACEMENT_3D ( 'NONE', #105704, #63842, #85408 ) ;
#88371=CARTESIAN_POINT ( 'NONE',  ( -12.69999999999999041, 12.50000000000000000, 3.983716857408420964 ) ) ;
#88372=CARTESIAN_POINT ( 'NONE',  ( -1.250000000000035749, 2.500000000000000000, -2.757883832488654097 ) ) ;
#88373=CIRCLE ( 'NONE', #48705, 0.06509327318403745899 ) ;
#88374=CIRCLE ( 'NONE', #90545, 0.06509327318403745899 ) ;
#88375=EDGE_LOOP ( 'NONE', ( #95277, #2532, #94953, #112382 ) ) ;
#88376=VECTOR ( 'NONE', #93313, 1000.000000000000000 ) ;
#88377=ADVANCED_FACE ( 'NONE', ( #29703 ), #56732, .T. ) ;
#88378=CARTESIAN_POINT ( 'NONE',  ( 12.89999999999990266, 12.50000000000000000, -3.637306695894650055 ) ) ;
#88379=CARTESIAN_POINT ( 'NONE',  ( -14.14999999999998614, 2.500000000000000000, 2.165063509461101265 ) ) ;
#88380=DIRECTION ( 'NONE',  ( 0.000000000000000000, 0.000000000000000000, -1.000000000000000000 ) ) ;
#88381=VECTOR ( 'NONE', #30654, 1000.000000000000000 ) ;
#88382=CARTESIAN_POINT ( 'NONE',  ( -11.84999999999999787, 12.50000000000000000, -6.148780366869522673 ) ) ;
#88383=AXIS2_PLACEMENT_3D ( 'NONE', #127977, #61174, #29154 ) ;
#88384=ORIENTED_EDGE ( 'NONE', *, *, #8145, .F. ) ;
#88385=DIRECTION ( 'NONE',  ( 0.000000000000000000, 1.000000000000000000, 0.000000000000000000 ) ) ;
#88386=EDGE_LOOP ( 'NONE', ( #64812, #86124 ) ) ;
#88387=CARTESIAN_POINT ( 'NONE',  ( -12.29999999999999538, 12.50000000000000000, -0.3464101615137741841 ) ) ;
#88388=AXIS2_PLACEMENT_3D ( 'NONE', #29876, #29247, #8925 ) ;
#88389=ORIENTED_EDGE ( 'NONE', *, *, #1494, .T. ) ;
#88390=DIRECTION ( 'NONE',  ( 0.000000000000000000, 0.000000000000000000, 1.000000000000000000 ) ) ;
#88391=CARTESIAN_POINT ( 'NONE',  ( 87.50000000000002842, -6.099025433955696407, 4.412011999988003197 ) ) ;
#88392=DIRECTION ( 'NONE',  ( 0.000000000000000000, 0.000000000000000000, -1.000000000000000000 ) ) ;
#88393=DIRECTION ( 'NONE',  ( 0.000000000000000000, 0.000000000000000000, 1.000000000000000000 ) ) ;
#88394=VERTEX_POINT ( 'NONE', #32313 ) ;
#88396=LINE ( 'NONE', #129019, #73153 ) ;
#88397=CARTESIAN_POINT ( 'NONE',  ( 87.50000000000001421, 3.974992050023852475, -6.359987280038158275 ) ) ;
#88398=EDGE_CURVE ( 'NONE', #8342, #94677, #119442, .T. ) ;
#88399=EDGE_CURVE ( 'NONE', #113969, #39135, #46289, .T. ) ;
#88400=FACE_OUTER_BOUND ( 'NONE', #29140, .T. ) ;
#88401=CARTESIAN_POINT ( 'NONE',  ( 10.19999999999991047, 12.50000000000000000, -4.048810130592463530 ) ) ;
#88402=ADVANCED_FACE ( 'NONE', ( #13912 ), #27491, .T. ) ;
#88403=EDGE_CURVE ( 'NONE', #88678, #99143, #72218, .T. ) ;
#88404=FACE_OUTER_BOUND ( 'NONE', #101933, .T. ) ;
#88405=CONICAL_SURFACE ( 'NONE', #25622, 0.1000000000000002554, 0.003490658503988666988 ) ;
#88406=ORIENTED_EDGE ( 'NONE', *, *, #5469, .T. ) ;
#88407=ORIENTED_EDGE ( 'NONE', *, *, #11623, .F. ) ;
#88408=FACE_OUTER_BOUND ( 'NONE', #106837, .T. ) ;
#88409=ADVANCED_FACE ( 'NONE', ( #102317 ), #102946, .T. ) ;
#88410=VERTEX_POINT ( 'NONE', #123244 ) ;
#88411=DIRECTION ( 'NONE',  ( 0.000000000000000000, 0.000000000000000000, 1.000000000000000000 ) ) ;
#88412=VERTEX_POINT ( 'NONE', #112137 ) ;
#88413=ORIENTED_EDGE ( 'NONE', *, *, #65041, .F. ) ;
#88414=ORIENTED_EDGE ( 'NONE', *, *, #54698, .F. ) ;
#88415=ADVANCED_FACE ( 'NONE', ( #73478 ), #122600, .T. ) ;
#88417=AXIS2_PLACEMENT_3D ( 'NONE', #2849, #73514, #23789 ) ;
#88418=AXIS2_PLACEMENT_3D ( 'NONE', #13354, #80830, #41559 ) ;
#88419=EDGE_CURVE ( 'NONE', #112572, #1361, #29671, .T. ) ;
#88421=CIRCLE ( 'NONE', #4787, 0.06509327318403743123 ) ;
#88422=EDGE_CURVE ( 'NONE', #51142, #62518, #83326, .T. ) ;
#88423=DIRECTION ( 'NONE',  ( 0.000000000000000000, -0.9999939076577903929, 0.003490651415223739937 ) ) ;
#88424=CARTESIAN_POINT ( 'NONE',  ( -4.800000000000026468, 12.50000000000000000, -4.741630453620016006 ) ) ;
#88425=DIRECTION ( 'NONE',  ( 0.000000000000000000, 1.000000000000000000, 0.000000000000000000 ) ) ;
#88426=CARTESIAN_POINT ( 'NONE',  ( -6.900000000000015454, 12.50000000000000000, 4.676537180435972552 ) ) ;
#88427=DIRECTION ( 'NONE',  ( -0.000000000000000000, -1.000000000000000000, -0.000000000000000000 ) ) ;
#88429=EDGE_CURVE ( 'NONE', #31342, #96613, #113416, .T. ) ;
#88430=AXIS2_PLACEMENT_3D ( 'NONE', #114055, #122586, #25028 ) ;
#88431=CARTESIAN_POINT ( 'NONE',  ( 8.749999999999921840, 2.500000000000000000, 2.757883832488649656 ) ) ;
#88432=VERTEX_POINT ( 'NONE', #72851 ) ;
#88433=AXIS2_PLACEMENT_3D ( 'NONE', #1313, #26, #9207 ) ;
#88434=VERTEX_POINT ( 'NONE', #52559 ) ;
#88435=CIRCLE ( 'NONE', #54989, 0.09999999999999982514 ) ;
#88436=ORIENTED_EDGE ( 'NONE', *, *, #90029, .T. ) ;
#88437=DIRECTION ( 'NONE',  ( -0.000000000000000000, -1.000000000000000000, -0.000000000000000000 ) ) ;
#88438=ORIENTED_EDGE ( 'NONE', *, *, #88179, .T. ) ;
#88439=ORIENTED_EDGE ( 'NONE', *, *, #77075, .F. ) ;
#88440=CARTESIAN_POINT ( 'NONE',  ( -1.850000000000033840, 2.500000000000000000, 1.818653347947321475 ) ) ;
#88441=DIRECTION ( 'NONE',  ( 0.000000000000000000, 0.000000000000000000, 1.000000000000000000 ) ) ;
#88442=CARTESIAN_POINT ( 'NONE',  ( -1.250000000000001110, 2.500000000000000000, -2.265063509461101798 ) ) ;
#88444=FACE_OUTER_BOUND ( 'NONE', #11514, .T. ) ;
#88445=CIRCLE ( 'NONE', #50903, 0.1000000000000002554 ) ;
#88446=CIRCLE ( 'NONE', #105176, 0.06509327318403745899 ) ;
#88447=DIRECTION ( 'NONE',  ( 0.000000000000000000, 1.000000000000000000, 0.000000000000000000 ) ) ;
#88448=ORIENTED_EDGE ( 'NONE', *, *, #49356, .T. ) ;
#88449=DIRECTION ( 'NONE',  ( 0.000000000000000000, 1.000000000000000000, 0.000000000000000000 ) ) ;
#88450=ORIENTED_EDGE ( 'NONE', *, *, #53880, .T. ) ;
#88451=CARTESIAN_POINT ( 'NONE',  ( 0.6499999999999561684, 2.500000000000000000, 2.511473670974873507 ) ) ;
#88452=EDGE_LOOP ( 'NONE', ( #123433, #118432 ) ) ;
#88453=CIRCLE ( 'NONE', #32054, 0.1000000000000002554 ) ;
#88454=DIRECTION ( 'NONE',  ( 0.000000000000000000, 0.000000000000000000, -1.000000000000000000 ) ) ;
#88455=ORIENTED_EDGE ( 'NONE', *, *, #114042, .T. ) ;
#88456=ORIENTED_EDGE ( 'NONE', *, *, #94317, .T. ) ;
#88457=CARTESIAN_POINT ( 'NONE',  ( 4.349999999999936584, 2.500000000000000000, 6.148780366869520009 ) ) ;
#88458=CARTESIAN_POINT ( 'NONE',  ( 59.86274543073836440, -3.775833904478944181, -4.995381933851996692 ) ) ;
#88459=EDGE_CURVE ( 'NONE', #47201, #10577, #53858, .T. ) ;
#88460=CARTESIAN_POINT ( 'NONE',  ( 6.899999999999928413, 2.500000000000000000, 3.883716857408421319 ) ) ;
#88461=PLANE ( 'NONE',  #547 ) ;
#88462=EDGE_CURVE ( 'NONE', #108826, #28226, #38078, .T. ) ;
#88463=DIRECTION ( 'NONE',  ( -4.274815082592931898E-19, -0.9999939076577903929, -0.003490651415223739937 ) ) ;
#88464=ORIENTED_EDGE ( 'NONE', *, *, #37237, .T. ) ;
#88465=CARTESIAN_POINT ( 'NONE',  ( 3.349999999999945466, 12.50000000000000000, -2.857883832488653741 ) ) ;
#88466=CARTESIAN_POINT ( 'NONE',  ( 8.549999999999924327, 2.500000000000000000, -6.941600689897077459 ) ) ;
#88467=AXIS2_PLACEMENT_3D ( 'NONE', #127570, #57545, #17600 ) ;
#88468=VECTOR ( 'NONE', #112563, 1000.000000000000000 ) ;
#88469=PLANE ( 'NONE',  #16453 ) ;
#88470=DIRECTION ( 'NONE',  ( -0.000000000000000000, 1.000000000000000000, -0.000000000000000000 ) ) ;
#88471=ADVANCED_FACE ( 'NONE', ( #123866 ), #88123, .T. ) ;
#88472=DIRECTION ( 'NONE',  ( 0.000000000000000000, -0.000000000000000000, 1.000000000000000000 ) ) ;
#88473=EDGE_LOOP ( 'NONE', ( #45025, #9693 ) ) ;
#88474=CIRCLE ( 'NONE', #32071, 0.1000000000000002554 ) ;
#88475=CIRCLE ( 'NONE', #117705, 0.06509327318403745899 ) ;
#88476=ORIENTED_EDGE ( 'NONE', *, *, #62198, .F. ) ;
#88477=AXIS2_PLACEMENT_3D ( 'NONE', #24834, #15636, #55584 ) ;
#88478=VECTOR ( 'NONE', #121963, 1000.000000000000000 ) ;
#88479=LINE ( 'NONE', #49876, #73822 ) ;
#88480=ORIENTED_EDGE ( 'NONE', *, *, #11658, .T. ) ;
#88481=CARTESIAN_POINT ( 'NONE',  ( 16.73738517751860755, -0.6985710796761546160, 5.899868569706077537 ) ) ;
#88482=DIRECTION ( 'NONE',  ( 0.000000000000000000, 0.000000000000000000, 1.000000000000000000 ) ) ;
#88484=AXIS2_PLACEMENT_3D ( 'NONE', #41024, #103139, #111003 ) ;
#88485=VECTOR ( 'NONE', #70300, 1000.000000000000000 ) ;
#88486=B_SPLINE_CURVE_WITH_KNOTS ( 'NONE', 3,
 ( #42990, #112349, #10890, #82896, #101235, #80318, #12191, #122811, #53435, #102520, #52141, #93351, #22046, #11553, #70482, #73067, #110403, #101883 ),
 .UNSPECIFIED., .F., .F.,
 ( 4, 2, 2, 2, 2, 2, 2, 2, 4 ),
 ( -1.046607274944176980E-05, 0.0004931538261971517897, 0.0009967737251437452407, 0.002004013523036937781, 0.002507633421983534484, 0.002759443371456834354, 0.003011253320930134657, 0.003514873219876733096, 0.004018493118823331968 ),
 .UNSPECIFIED. ) ;
#88487=AXIS2_PLACEMENT_3D ( 'NONE', #52215, #63313, #22130 ) ;
#88488=AXIS2_PLACEMENT_3D ( 'NONE', #76068, #127736, #38074 ) ;
#88489=EDGE_LOOP ( 'NONE', ( #80005, #10462, #106919, #66960 ) ) ;
#88491=LINE ( 'NONE', #128450, #22383 ) ;
#88492=CARTESIAN_POINT ( 'NONE',  ( 8.149999999999920419, 12.50000000000000000, 6.148780366869520897 ) ) ;
#88493=DIRECTION ( 'NONE',  ( -0.000000000000000000, 1.000000000000000000, -0.000000000000000000 ) ) ;
#88494=ORIENTED_EDGE ( 'NONE', *, *, #480, .F. ) ;
#88495=AXIS2_PLACEMENT_3D ( 'NONE', #106811, #28271, #6034 ) ;
#88496=DIRECTION ( 'NONE',  ( 0.000000000000000000, -0.000000000000000000, 1.000000000000000000 ) ) ;
#88497=ORIENTED_EDGE ( 'NONE', *, *, #29746, .F. ) ;
#88498=CARTESIAN_POINT ( 'NONE',  ( 48.67918707175899584, 3.179367830269037132, -5.083100937075674786 ) ) ;
#88499=PLANE ( 'NONE',  #129285 ) ;
#88500=DIRECTION ( 'NONE',  ( -0.000000000000000000, 1.000000000000000000, -0.000000000000000000 ) ) ;
#88501=AXIS2_PLACEMENT_3D ( 'NONE', #15900, #55835, #6075 ) ;
#88502=ORIENTED_EDGE ( 'NONE', *, *, #64494, .F. ) ;
#88503=CARTESIAN_POINT ( 'NONE',  ( -5.850000000000019185, 2.500000000000000000, 2.265063509461097357 ) ) ;
#88504=ORIENTED_EDGE ( 'NONE', *, *, #32600, .F. ) ;
#88505=CARTESIAN_POINT ( 'NONE',  ( 5.799999999999934985, 12.50000000000000000, -4.330127018922201643 ) ) ;
#88506=CARTESIAN_POINT ( 'NONE',  ( 10.79999999999991012, 12.50000000000000000, -4.265033745738164406 ) ) ;
#88507=DIRECTION ( 'NONE',  ( 0.000000000000000000, -0.000000000000000000, 1.000000000000000000 ) ) ;
#88508=AXIS2_PLACEMENT_3D ( 'NONE', #105891, #33930, #52928 ) ;
#88509=ORIENTED_EDGE ( 'NONE', *, *, #68407, .F. ) ;
#88510=CONICAL_SURFACE ( 'NONE', #69743, 0.1000000000000000472, 0.003490658503988666988 ) ;
#88511=CARTESIAN_POINT ( 'NONE',  ( -2.500000000000032419, 12.50000000000000000, 0.6928203230275494784 ) ) ;
#88514=ORIENTED_EDGE ( 'NONE', *, *, #32433, .T. ) ;
#88515=CARTESIAN_POINT ( 'NONE',  ( -0.6500000000000403233, 12.50000000000000000, 1.818653347947321475 ) ) ;
#88516=EDGE_CURVE ( 'NONE', #120717, #44822, #127865, .T. ) ;
#88517=AXIS2_PLACEMENT_3D ( 'NONE', #33964, #73883, #103994 ) ;
#88518=ORIENTED_EDGE ( 'NONE', *, *, #110702, .F. ) ;
#88519=AXIS2_PLACEMENT_3D ( 'NONE', #51606, #22800, #123538 ) ;
#88520=DIRECTION ( 'NONE',  ( 0.000000000000000000, 0.000000000000000000, -1.000000000000000000 ) ) ;
#88521=VECTOR ( 'NONE', #46897, 1000.000000000000000 ) ;
#88522=AXIS2_PLACEMENT_3D ( 'NONE', #54364, #2670, #93016 ) ;
#88523=ORIENTED_EDGE ( 'NONE', *, *, #39975, .F. ) ;
#88524=DIRECTION ( 'NONE',  ( -4.274815082592931898E-19, -0.9999939076577903929, -0.003490651415223739937 ) ) ;
#88525=CARTESIAN_POINT ( 'NONE',  ( 10.44999999999991402, 12.50000000000000000, -2.165063509461101710 ) ) ;
#88526=ORIENTED_EDGE ( 'NONE', *, *, #55259, .T. ) ;
#88527=ADVANCED_FACE ( 'NONE', ( #53222 ), #119536, .T. ) ;
#88528=ORIENTED_EDGE ( 'NONE', *, *, #39541, .F. ) ;
#88529=CIRCLE ( 'NONE', #27905, 0.06509327318403745899 ) ;
#88530=LINE ( 'NONE', #96408, #86493 ) ;
#88531=DIRECTION ( 'NONE',  ( -0.000000000000000000, -1.000000000000000000, -0.000000000000000000 ) ) ;
#88532=ORIENTED_EDGE ( 'NONE', *, *, #43252, .T. ) ;
#88533=DIRECTION ( 'NONE',  ( -0.000000000000000000, 1.000000000000000000, -0.000000000000000000 ) ) ;
#88534=CARTESIAN_POINT ( 'NONE',  ( 21.24754738303277435, 0.7337760880902381988, 4.182111650399361835 ) ) ;
#88535=AXIS2_PLACEMENT_3D ( 'NONE', #89959, #103668, #13969 ) ;
#88536=DIRECTION ( 'NONE',  ( -0.000000000000000000, 1.000000000000000000, -0.000000000000000000 ) ) ;
#88537=AXIS2_PLACEMENT_3D ( 'NONE', #76877, #54016, #84763 ) ;
#88538=VECTOR ( 'NONE', #81661, 1000.000000000000000 ) ;
#88540=DIRECTION ( 'NONE',  ( 0.000000000000000000, 0.000000000000000000, 1.000000000000000000 ) ) ;
#88541=CARTESIAN_POINT ( 'NONE',  ( 6.249999999999930722, 2.500000000000000000, 1.472243186433545459 ) ) ;
#88542=VECTOR ( 'NONE', #105782, 1000.000000000000000 ) ;
#88543=DIRECTION ( 'NONE',  ( 0.000000000000000000, 1.000000000000000000, 0.000000000000000000 ) ) ;
#88544=AXIS2_PLACEMENT_3D ( 'NONE', #13983, #5453, #4803 ) ;
#88545=ORIENTED_EDGE ( 'NONE', *, *, #98026, .F. ) ;
#88546=EDGE_CURVE ( 'NONE', #91772, #108234, #23394, .T. ) ;
#88547=ORIENTED_EDGE ( 'NONE', *, *, #82078, .F. ) ;
#88548=EDGE_LOOP ( 'NONE', ( #116973, #99162 ) ) ;
#88549=EDGE_LOOP ( 'NONE', ( #50675, #40801, #111033, #1218 ) ) ;
#88550=CARTESIAN_POINT ( 'NONE',  ( -8.350000000000013856, 2.500000000000000000, 2.165063509461097713 ) ) ;
#88551=CARTESIAN_POINT ( 'NONE',  ( 5.849999999999933920, 12.50000000000000000, -2.857883832488653741 ) ) ;
#88552=DIRECTION ( 'NONE',  ( -4.274815082592931898E-19, -0.9999939076577903929, -0.003490651415223739937 ) ) ;
#88553=ORIENTED_EDGE ( 'NONE', *, *, #65098, .F. ) ;
#88554=FACE_BOUND ( 'NONE', #52429, .T. ) ;
#88555=ORIENTED_EDGE ( 'NONE', *, *, #119478, .T. ) ;
#88556=DIRECTION ( 'NONE',  ( 0.000000000000000000, 0.000000000000000000, -1.000000000000000000 ) ) ;
#88557=CARTESIAN_POINT ( 'NONE',  ( -4.200000000000025935, 2.500000000000000000, -2.385244779468109755E-15 ) ) ;
#88558=CARTESIAN_POINT ( 'NONE',  ( -8.100000000000013856, 12.50000000000000000, -0.2813168883297408329 ) ) ;
#88559=EDGE_CURVE ( 'NONE', #91737, #33523, #79835, .T. ) ;
#88560=CARTESIAN_POINT ( 'NONE',  ( -6.250000000000015987, 2.500000000000000000, 5.802370205355744659 ) ) ;
#88561=LINE ( 'NONE', #60427, #98803 ) ;
#88562=DIRECTION ( 'NONE',  ( -0.000000000000000000, -1.000000000000000000, -0.000000000000000000 ) ) ;
#88563=DIRECTION ( 'NONE',  ( 0.000000000000000000, 0.000000000000000000, 1.000000000000000000 ) ) ;
#88564=CARTESIAN_POINT ( 'NONE',  ( 14.99999999999989342, 12.50000000000000000, -0.6928203230275541413 ) ) ;
#88565=CIRCLE ( 'NONE', #25875, 0.1000000000000002554 ) ;
#88566=EDGE_CURVE ( 'NONE', #127598, #92529, #66881, .T. ) ;
#88567=CIRCLE ( 'NONE', #101089, 0.1000000000000002554 ) ;
#88568=EDGE_CURVE ( 'NONE', #66767, #74569, #107007, .T. ) ;
#88569=DIRECTION ( 'NONE',  ( 0.000000000000000000, 0.000000000000000000, 1.000000000000000000 ) ) ;
#88570=ADVANCED_FACE ( 'NONE', ( #37447 ), #74789, .T. ) ;
#88571=EDGE_CURVE ( 'NONE', #119467, #101350, #15189, .T. ) ;
#88572=DIRECTION ( 'NONE',  ( -0.000000000000000000, -1.000000000000000000, -0.000000000000000000 ) ) ;
#88573=CONICAL_SURFACE ( 'NONE', #71865, 0.1000000000000002554, 0.003490658503988666988 ) ;
#88574=EDGE_LOOP ( 'NONE', ( #87664, #98872 ) ) ;
#88575=ORIENTED_EDGE ( 'NONE', *, *, #117108, .F. ) ;
#88576=ORIENTED_EDGE ( 'NONE', *, *, #13238, .T. ) ;
#88577=AXIS2_PLACEMENT_3D ( 'NONE', #40444, #19483, #101276 ) ;
#88578=ORIENTED_EDGE ( 'NONE', *, *, #68646, .T. ) ;
#88579=CARTESIAN_POINT ( 'NONE',  ( 17.41715230668671310, -1.872943439149598710, -4.643388583737356079 ) ) ;
#88580=EDGE_CURVE ( 'NONE', #113146, #117732, #12918, .T. ) ;
#88581=AXIS2_PLACEMENT_3D ( 'NONE', #110838, #11359, #111487 ) ;
#88582=CARTESIAN_POINT ( 'NONE',  ( 9.149999999999920419, 12.50000000000000000, -5.802370205355749988 ) ) ;
#88583=ADVANCED_FACE ( 'NONE', ( #54488 ), #6637, .T. ) ;
#88584=ORIENTED_EDGE ( 'NONE', *, *, #19427, .F. ) ;
#88585=ORIENTED_EDGE ( 'NONE', *, *, #14129, .T. ) ;
#88588=AXIS2_PLACEMENT_3D ( 'NONE', #1881, #92863, #62755 ) ;
#88589=ADVANCED_FACE ( 'NONE', ( #5388 ), #96996, .T. ) ;
#88590=AXIS2_PLACEMENT_3D ( 'NONE', #115284, #14383, #124366 ) ;
#88591=CIRCLE ( 'NONE', #94847, 0.1000000000000002554 ) ;
#88592=EDGE_CURVE ( 'NONE', #80576, #53022, #94407, .T. ) ;
#88593=DIRECTION ( 'NONE',  ( 0.000000000000000000, 1.000000000000000000, 0.000000000000000000 ) ) ;
#88594=CARTESIAN_POINT ( 'NONE',  ( -4.150000000000027889, 2.500000000000000000, -6.495190528383302464 ) ) ;
#88595=CARTESIAN_POINT ( 'NONE',  ( -7.950000000000012612, 12.50000000000000000, -2.099970236277064473 ) ) ;
#88596=LINE ( 'NONE', #28394, #26266 ) ;
#88597=DIRECTION ( 'NONE',  ( 0.000000000000000000, 0.000000000000000000, 1.000000000000000000 ) ) ;
#88598=AXIS2_PLACEMENT_3D ( 'NONE', #25499, #62872, #65433 ) ;
#88599=DIRECTION ( 'NONE',  ( 0.000000000000000000, 0.000000000000000000, -1.000000000000000000 ) ) ;
#88600=ORIENTED_EDGE ( 'NONE', *, *, #41795, .F. ) ;
#88601=ADVANCED_FACE ( 'NONE', ( #56419 ), #125173, .T. ) ;
#88602=DIRECTION ( 'NONE',  ( 0.000000000000000000, 0.000000000000000000, 1.000000000000000000 ) ) ;
#88603=ORIENTED_EDGE ( 'NONE', *, *, #3868, .T. ) ;
#88604=ORIENTED_EDGE ( 'NONE', *, *, #88546, .T. ) ;
#88605=VERTEX_POINT ( 'NONE', #4724 ) ;
#88606=DIRECTION ( 'NONE',  ( 0.000000000000000000, 0.000000000000000000, 1.000000000000000000 ) ) ;
#88607=VERTEX_POINT ( 'NONE', #7313 ) ;
#88608=ORIENTED_EDGE ( 'NONE', *, *, #45608, .F. ) ;
#88609=CIRCLE ( 'NONE', #9092, 0.1000000000000002554 ) ;
#88610=DIRECTION ( 'NONE',  ( 0.000000000000000000, 0.000000000000000000, 1.000000000000000000 ) ) ;
#88611=FACE_OUTER_BOUND ( 'NONE', #122838, .T. ) ;
#88612=CARTESIAN_POINT ( 'NONE',  ( -10.00000000000000533, 12.50000000000000000, -5.088040615133786915 ) ) ;
#88613=DIRECTION ( 'NONE',  ( 0.000000000000000000, 0.000000000000000000, 1.000000000000000000 ) ) ;
#88614=DIRECTION ( 'NONE',  ( 0.000000000000000000, 1.000000000000000000, 0.000000000000000000 ) ) ;
#88615=VECTOR ( 'NONE', #85444, 1000.000000000000000 ) ;
#88616=ORIENTED_EDGE ( 'NONE', *, *, #74885, .F. ) ;
#88617=FACE_OUTER_BOUND ( 'NONE', #102010, .T. ) ;
#88618=AXIS2_PLACEMENT_3D ( 'NONE', #43330, #124456, #44605 ) ;
#88619=VECTOR ( 'NONE', #104143, 1000.000000000000000 ) ;
#88620=ORIENTED_EDGE ( 'NONE', *, *, #9037, .F. ) ;
#88621=CARTESIAN_POINT ( 'NONE',  ( 21.25104915410168971, -0.2454763298545039607, 4.189301388122809833 ) ) ;
#88622=EDGE_LOOP ( 'NONE', ( #68824, #5569 ) ) ;
#88624=FACE_OUTER_BOUND ( 'NONE', #97062, .T. ) ;
#88625=EDGE_LOOP ( 'NONE', ( #96631, #70963, #128240, #26064 ) ) ;
#88628=ORIENTED_EDGE ( 'NONE', *, *, #120342, .F. ) ;
#88629=AXIS2_PLACEMENT_3D ( 'NONE', #85990, #86656, #95840 ) ;
#88630=CIRCLE ( 'NONE', #99107, 0.06509327318403745899 ) ;
#88631=EDGE_CURVE ( 'NONE', #58954, #128192, #73561, .T. ) ;
#88632=DIRECTION ( 'NONE',  ( -0.000000000000000000, 1.000000000000000000, -0.000000000000000000 ) ) ;
#88633=EDGE_CURVE ( 'NONE', #71810, #4409, #10854, .T. ) ;
#88634=EDGE_LOOP ( 'NONE', ( #107835, #14714, #57092, #68173 ) ) ;
#88635=ORIENTED_EDGE ( 'NONE', *, *, #11478, .T. ) ;
#88636=DIRECTION ( 'NONE',  ( 0.000000000000000000, 0.000000000000000000, 1.000000000000000000 ) ) ;
#88637=DIRECTION ( 'NONE',  ( 0.000000000000000000, 0.000000000000000000, 1.000000000000000000 ) ) ;
#88638=DIRECTION ( 'NONE',  ( -0.000000000000000000, -1.000000000000000000, -0.000000000000000000 ) ) ;
#88639=CARTESIAN_POINT ( 'NONE',  ( 6.649999999999930189, 2.500000000000000000, -2.857883832488653741 ) ) ;
#88640=PLANE ( 'NONE',  #43726 ) ;
#88641=ORIENTED_EDGE ( 'NONE', *, *, #109988, .T. ) ;
#88642=AXIS2_PLACEMENT_3D ( 'NONE', #67579, #107522, #78059 ) ;
#88643=AXIS2_PLACEMENT_3D ( 'NONE', #91616, #13033, #41892 ) ;
#88644=AXIS2_PLACEMENT_3D ( 'NONE', #50139, #41612, #90025 ) ;
#88645=CARTESIAN_POINT ( 'NONE',  ( 8.549999999999920774, 12.50000000000000000, -2.446380397790840266 ) ) ;
#88646=AXIS2_PLACEMENT_3D ( 'NONE', #34329, #104954, #46067 ) ;
#88647=EDGE_LOOP ( 'NONE', ( #77273, #11924 ) ) ;
#88648=CONICAL_SURFACE ( 'NONE', #38499, 0.09999999999999982514, 0.003490658503988666988 ) ;
#88649=LINE ( 'NONE', #29104, #111311 ) ;
#88650=DIRECTION ( 'NONE',  ( 0.000000000000000000, 0.000000000000000000, -1.000000000000000000 ) ) ;
#88651=ORIENTED_EDGE ( 'NONE', *, *, #102290, .T. ) ;
#88652=DIRECTION ( 'NONE',  ( 0.000000000000000000, -0.000000000000000000, 1.000000000000000000 ) ) ;
#88654=PLANE ( 'NONE',  #67367 ) ;
#88655=DIRECTION ( 'NONE',  ( 0.000000000000000000, 0.000000000000000000, 1.000000000000000000 ) ) ;
#88656=CARTESIAN_POINT ( 'NONE',  ( 14.59999999999989484, 2.500000000000000000, 0.7928203230275495672 ) ) ;
#88657=VERTEX_POINT ( 'NONE', #115316 ) ;
#88658=CARTESIAN_POINT ( 'NONE',  ( 11.04999999999991012, 2.500000000000000000, -1.918653347947326004 ) ) ;
#88659=CARTESIAN_POINT ( 'NONE',  ( -5.400000000000019895, 2.500000000000000000, 0.09999999999999772959 ) ) ;
#88660=DIRECTION ( 'NONE',  ( 0.000000000000000000, 0.000000000000000000, 1.000000000000000000 ) ) ;
#88661=CIRCLE ( 'NONE', #126321, 0.06509327318403745899 ) ;
#88662=VECTOR ( 'NONE', #71072, 1000.000000000000000 ) ;
#88663=AXIS2_PLACEMENT_3D ( 'NONE', #121560, #52837, #61376 ) ;
#88664=ORIENTED_EDGE ( 'NONE', *, *, #4672, .T. ) ;
#88665=CARTESIAN_POINT ( 'NONE',  ( -2.300000000000032685, 2.500000000000000000, -0.2464101615137783419 ) ) ;
#88666=ADVANCED_FACE ( 'NONE', ( #25039 ), #14955, .T. ) ;
#88667=AXIS2_PLACEMENT_3D ( 'NONE', #57116, #106229, #46663 ) ;
#88668=AXIS2_PLACEMENT_3D ( 'NONE', #71091, #110989, #20706 ) ;
#88669=VERTEX_POINT ( 'NONE', #127117 ) ;
#88670=CIRCLE ( 'NONE', #111667, 0.1000000000000000472 ) ;
#88671=ORIENTED_EDGE ( 'NONE', *, *, #15461, .F. ) ;
#88672=CARTESIAN_POINT ( 'NONE',  ( -13.09999999999999076, 2.500000000000000000, 4.776537180435972196 ) ) ;
#88673=CONICAL_SURFACE ( 'NONE', #92798, 0.1000000000000002554, 0.003490658503988666988 ) ;
#88674=VERTEX_POINT ( 'NONE', #15847 ) ;
#88676=FACE_OUTER_BOUND ( 'NONE', #98553, .T. ) ;
#88677=AXIS2_PLACEMENT_3D ( 'NONE', #67211, #8318, #46982 ) ;
#88678=VERTEX_POINT ( 'NONE', #25673 ) ;
#88679=AXIS2_PLACEMENT_3D ( 'NONE', #22805, #70596, #12939 ) ;
#88680=CARTESIAN_POINT ( 'NONE',  ( -8.750000000000010658, 2.500000000000000000, -7.188010851410848723 ) ) ;
#88681=DIRECTION ( 'NONE',  ( 0.000000000000000000, 1.000000000000000000, 0.000000000000000000 ) ) ;
#88682=ORIENTED_EDGE ( 'NONE', *, *, #53824, .F. ) ;
#88683=AXIS2_PLACEMENT_3D ( 'NONE', #69292, #111824, #99433 ) ;
#88684=EDGE_CURVE ( 'NONE', #93998, #118854, #36803, .T. ) ;
#88685=DIRECTION ( 'NONE',  ( 0.000000000000000000, 1.000000000000000000, 0.000000000000000000 ) ) ;
#88686=CARTESIAN_POINT ( 'NONE',  ( -2.300000000000032685, 2.500000000000000000, -4.576537180435978236 ) ) ;
#88687=EDGE_CURVE ( 'NONE', #78285, #93896, #86072, .T. ) ;
#88688=VERTEX_POINT ( 'NONE', #124536 ) ;
#88689=ORIENTED_EDGE ( 'NONE', *, *, #127338, .F. ) ;
#88690=VERTEX_POINT ( 'NONE', #55785 ) ;
#88691=FACE_OUTER_BOUND ( 'NONE', #114179, .T. ) ;
#88692=DIRECTION ( 'NONE',  ( -0.000000000000000000, -1.000000000000000000, -0.000000000000000000 ) ) ;
#88693=DIRECTION ( 'NONE',  ( -0.000000000000000000, -1.000000000000000000, -0.000000000000000000 ) ) ;
#88694=ADVANCED_FACE ( 'NONE', ( #45979 ), #85867, .T. ) ;
#88695=FACE_BOUND ( 'NONE', #80758, .T. ) ;
#88696=ORIENTED_EDGE ( 'NONE', *, *, #107874, .F. ) ;
#88697=DIRECTION ( 'NONE',  ( -4.274815082592931898E-19, -0.9999939076577903929, -0.003490651415223739937 ) ) ;
#88698=CARTESIAN_POINT ( 'NONE',  ( -9.350000000000006750, 2.500000000000000000, -1.718653347947325827 ) ) ;
#88699=AXIS2_PLACEMENT_3D ( 'NONE', #70024, #128309, #79829 ) ;
#88700=VERTEX_POINT ( 'NONE', #129060 ) ;
#88701=DIRECTION ( 'NONE',  ( 0.000000000000000000, -0.9999939076577903929, 0.003490651415223739937 ) ) ;
#88702=DIRECTION ( 'NONE',  ( 0.000000000000000000, 1.000000000000000000, 0.000000000000000000 ) ) ;
#88703=DIRECTION ( 'NONE',  ( 0.000000000000000000, 0.000000000000000000, 1.000000000000000000 ) ) ;
#88704=CARTESIAN_POINT ( 'NONE',  ( 5.449999999999936229, 12.50000000000000000, 6.495190528383297135 ) ) ;
#88705=DIRECTION ( 'NONE',  ( 0.000000000000000000, 0.000000000000000000, 1.000000000000000000 ) ) ;
#88706=CARTESIAN_POINT ( 'NONE',  ( 3.149999999999942624, 2.500000000000000000, 6.148780366869520897 ) ) ;
#88707=CARTESIAN_POINT ( 'NONE',  ( -6.083778633910298187E-15, 2.500000000000000000, -4.430127018922202176 ) ) ;
#88708=CIRCLE ( 'NONE', #34354, 0.1000000000000000472 ) ;
#88709=AXIS2_PLACEMENT_3D ( 'NONE', #41862, #81759, #121686 ) ;
#88710=VERTEX_POINT ( 'NONE', #118561 ) ;
#88711=ORIENTED_EDGE ( 'NONE', *, *, #41935, .T. ) ;
#88712=ORIENTED_EDGE ( 'NONE', *, *, #83322, .F. ) ;
#88713=VERTEX_POINT ( 'NONE', #90377 ) ;
#88714=ORIENTED_EDGE ( 'NONE', *, *, #76440, .F. ) ;
#88715=CARTESIAN_POINT ( 'NONE',  ( -1.450000000000035927, 2.500000000000000000, -6.148780366869526226 ) ) ;
#88716=DIRECTION ( 'NONE',  ( 0.000000000000000000, 1.000000000000000000, 0.000000000000000000 ) ) ;
#88718=FACE_BOUND ( 'NONE', #129047, .T. ) ;
#88719=FACE_OUTER_BOUND ( 'NONE', #47565, .T. ) ;
#88720=VECTOR ( 'NONE', #121341, 1000.000000000000000 ) ;
#88721=ADVANCED_FACE ( 'NONE', ( #110044 ), #77, .T. ) ;
#88722=CARTESIAN_POINT ( 'NONE',  ( 11.89999999999990443, 12.50000000000000000, 0.4115034346978110880 ) ) ;
#88723=DIRECTION ( 'NONE',  ( 0.000000000000000000, -0.9999939076577903929, 0.003490651415223739937 ) ) ;
#88724=DIRECTION ( 'NONE',  ( 0.000000000000000000, 0.000000000000000000, -1.000000000000000000 ) ) ;
#88725=EDGE_CURVE ( 'NONE', #95323, #69394, #42192, .T. ) ;
#88726=FACE_OUTER_BOUND ( 'NONE', #20738, .T. ) ;
#88727=ORIENTED_EDGE ( 'NONE', *, *, #111728, .T. ) ;
#88728=EDGE_CURVE ( 'NONE', #52632, #58166, #17105, .T. ) ;
#88729=ORIENTED_EDGE ( 'NONE', *, *, #41881, .T. ) ;
#88730=AXIS2_PLACEMENT_3D ( 'NONE', #96241, #83848, #84509 ) ;
#88731=ORIENTED_EDGE ( 'NONE', *, *, #52775, .T. ) ;
#88732=ORIENTED_EDGE ( 'NONE', *, *, #53995, .T. ) ;
#88733=ADVANCED_FACE ( 'NONE', ( #107461 ), #19179, .T. ) ;
#88734=CARTESIAN_POINT ( 'NONE',  ( 6.899999999999928413, 2.500000000000000000, -4.083716857408426826 ) ) ;
#88735=CARTESIAN_POINT ( 'NONE',  ( 3.677302434130802933, 2.500000000000000444, 9.000000000000007105 ) ) ;
#88736=EDGE_CURVE ( 'NONE', #61895, #63523, #63109, .T. ) ;
#88737=FACE_OUTER_BOUND ( 'NONE', #24042, .T. ) ;
#88738=AXIS2_PLACEMENT_3D ( 'NONE', #32243, #42712, #80029 ) ;
#88739=EDGE_CURVE ( 'NONE', #82776, #44898, #2458, .T. ) ;
#88740=EDGE_LOOP ( 'NONE', ( #20255, #10449 ) ) ;
#88741=FACE_OUTER_BOUND ( 'NONE', #14636, .T. ) ;
#88742=AXIS2_PLACEMENT_3D ( 'NONE', #74367, #77570, #107027 ) ;
#88743=CARTESIAN_POINT ( 'NONE',  ( 12.89999999999990088, 12.50000000000000000, -4.265033745738164406 ) ) ;
#88744=DIRECTION ( 'NONE',  ( -0.000000000000000000, -1.000000000000000000, -0.000000000000000000 ) ) ;
#88745=EDGE_CURVE ( 'NONE', #92207, #45669, #35920, .T. ) ;
#88747=DIRECTION ( 'NONE',  ( 0.000000000000000000, 1.000000000000000000, 0.000000000000000000 ) ) ;
#88748=CARTESIAN_POINT ( 'NONE',  ( 11.24999999999991118, 12.50000000000000000, 5.802370205355744659 ) ) ;
#88750=VERTEX_POINT ( 'NONE', #30211 ) ;
#88751=DIRECTION ( 'NONE',  ( 0.000000000000000000, 1.000000000000000000, 0.000000000000000000 ) ) ;
#88752=ADVANCED_FACE ( 'NONE', ( #70126 ), #52982, .T. ) ;
#88753=ORIENTED_EDGE ( 'NONE', *, *, #6841, .T. ) ;
#88754=CIRCLE ( 'NONE', #80639, 0.1000000000000002554 ) ;
#88755=ORIENTED_EDGE ( 'NONE', *, *, #19733, .T. ) ;
#88756=DIRECTION ( 'NONE',  ( -0.000000000000000000, 1.000000000000000000, -0.000000000000000000 ) ) ;
#88757=CIRCLE ( 'NONE', #49064, 0.06509327318403745899 ) ;
#88758=CARTESIAN_POINT ( 'NONE',  ( 0.1999999999999562961, 2.500000000000000000, 4.776537180435972196 ) ) ;
#88759=CONICAL_SURFACE ( 'NONE', #21876, 0.1000000000000000472, 0.003490658503988666988 ) ;
#88760=PLANE ( 'NONE',  #10648 ) ;
#88761=ORIENTED_EDGE ( 'NONE', *, *, #67449, .T. ) ;
#88762=EDGE_LOOP ( 'NONE', ( #10179, #79224, #85333, #18520 ) ) ;
#88764=VECTOR ( 'NONE', #26148, 1000.000000000000000 ) ;
#88765=AXIS2_PLACEMENT_3D ( 'NONE', #127058, #37392, #115260 ) ;
#88766=CIRCLE ( 'NONE', #105498, 0.1000000000000002554 ) ;
#88767=CARTESIAN_POINT ( 'NONE',  ( 8.349999999999919709, 2.500000000000000000, 6.395190528383296602 ) ) ;
#88768=CARTESIAN_POINT ( 'NONE',  ( 1.049999999999952083, 2.500000000000000000, 6.741600689897071952 ) ) ;
#88769=ORIENTED_EDGE ( 'NONE', *, *, #103066, .T. ) ;
#88770=ORIENTED_EDGE ( 'NONE', *, *, #30240, .F. ) ;
#88771=CONICAL_SURFACE ( 'NONE', #28426, 0.1000000000000002554, 0.003490658503988666988 ) ;
#88772=DIRECTION ( 'NONE',  ( 0.000000000000000000, 1.000000000000000000, 0.000000000000000000 ) ) ;
#88773=ORIENTED_EDGE ( 'NONE', *, *, #77914, .T. ) ;
#88774=DIRECTION ( 'NONE',  ( 0.000000000000000000, 1.000000000000000000, 0.000000000000000000 ) ) ;
#88775=AXIS2_PLACEMENT_3D ( 'NONE', #46278, #76399, #6975 ) ;
#88776=CIRCLE ( 'NONE', #28139, 0.06509327318403745899 ) ;
#88777=ORIENTED_EDGE ( 'NONE', *, *, #102232, .F. ) ;
#88778=CARTESIAN_POINT ( 'NONE',  ( 0.3999999999999619971, 2.500000000000000000, -1.084202172485504434E-16 ) ) ;
#88779=DIRECTION ( 'NONE',  ( 0.000000000000000000, -0.9999939076577903929, 0.003490651415223739937 ) ) ;
#88780=DIRECTION ( 'NONE',  ( -0.000000000000000000, -1.000000000000000000, -0.000000000000000000 ) ) ;
#88781=CONICAL_SURFACE ( 'NONE', #84575, 0.1000000000000002554, 0.003490658503988666988 ) ;
#88782=DIRECTION ( 'NONE',  ( 0.000000000000000000, 0.000000000000000000, -1.000000000000000000 ) ) ;
#88783=VERTEX_POINT ( 'NONE', #68170 ) ;
#88784=FACE_OUTER_BOUND ( 'NONE', #64191, .T. ) ;
#88785=ADVANCED_FACE ( 'NONE', ( #10533 ), #71866, .T. ) ;
#88786=VERTEX_POINT ( 'NONE', #50469 ) ;
#88787=ORIENTED_EDGE ( 'NONE', *, *, #97812, .F. ) ;
#88788=CARTESIAN_POINT ( 'NONE',  ( 0.5999999999999551248, 2.500000000000000000, -4.776537180435978414 ) ) ;
#88789=DIRECTION ( 'NONE',  ( 0.000000000000000000, 1.000000000000000000, 0.000000000000000000 ) ) ;
#88790=CARTESIAN_POINT ( 'NONE',  ( 12.89999999999990266, 12.50000000000000000, 3.637306695894644726 ) ) ;
#88791=DIRECTION ( 'NONE',  ( -0.000000000000000000, 1.000000000000000000, -0.000000000000000000 ) ) ;
#88792=CIRCLE ( 'NONE', #107575, 0.06509327318403745899 ) ;
#88793=DIRECTION ( 'NONE',  ( -0.000000000000000000, -1.000000000000000000, -0.000000000000000000 ) ) ;
#88794=PLANE ( 'NONE',  #115488 ) ;
#88795=EDGE_CURVE ( 'NONE', #124254, #1046, #21690, .T. ) ;
#88796=FACE_OUTER_BOUND ( 'NONE', #68650, .T. ) ;
#88797=DIRECTION ( 'NONE',  ( 0.000000000000000000, 0.000000000000000000, -1.000000000000000000 ) ) ;
#88798=DIRECTION ( 'NONE',  ( -0.000000000000000000, -1.000000000000000000, -0.000000000000000000 ) ) ;
#88799=VECTOR ( 'NONE', #77600, 1000.000000000000000 ) ;
#88800=AXIS2_PLACEMENT_3D ( 'NONE', #122833, #43643, #80978 ) ;
#88801=ORIENTED_EDGE ( 'NONE', *, *, #122307, .F. ) ;
#88802=CARTESIAN_POINT ( 'NONE',  ( 1.049999999999954081, 12.50000000000000000, -6.148780366869526226 ) ) ;
#88803=DIRECTION ( 'NONE',  ( 0.000000000000000000, 0.000000000000000000, -1.000000000000000000 ) ) ;
#88804=CARTESIAN_POINT ( 'NONE',  ( 3.749999999999978684, 2.500000000000000000, -6.595190528383302109 ) ) ;
#88805=CARTESIAN_POINT ( 'NONE',  ( -14.99999999999994671, 2.500000000000000000, 0.1000000000000000056 ) ) ;
#88806=DIRECTION ( 'NONE',  ( 0.000000000000000000, 0.000000000000000000, 1.000000000000000000 ) ) ;
#88807=EDGE_LOOP ( 'NONE', ( #74720, #23476, #83510, #115922 ) ) ;
#88808=DIRECTION ( 'NONE',  ( 0.000000000000000000, 0.000000000000000000, 1.000000000000000000 ) ) ;
#88809=AXIS2_PLACEMENT_3D ( 'NONE', #6068, #25719, #85287 ) ;
#88810=AXIS2_PLACEMENT_3D ( 'NONE', #12399, #61529, #22889 ) ;
#88811=DIRECTION ( 'NONE',  ( 0.000000000000000000, 1.000000000000000000, 0.000000000000000000 ) ) ;
#88812=DIRECTION ( 'NONE',  ( 0.000000000000000000, 0.000000000000000000, -1.000000000000000000 ) ) ;
#88813=ORIENTED_EDGE ( 'NONE', *, *, #39050, .T. ) ;
#88814=EDGE_LOOP ( 'NONE', ( #106228, #41769 ) ) ;
#88815=CARTESIAN_POINT ( 'NONE',  ( -13.94999999999998685, 2.500000000000000000, 1.718653347947325383 ) ) ;
#88816=EDGE_CURVE ( 'NONE', #101430, #110184, #59358, .T. ) ;
#88817=CIRCLE ( 'NONE', #17704, 0.06509327318403745899 ) ;
#88818=ORIENTED_EDGE ( 'NONE', *, *, #2929, .F. ) ;
#88819=VERTEX_POINT ( 'NONE', #40682 ) ;
#88820=ORIENTED_EDGE ( 'NONE', *, *, #121284, .T. ) ;
#88821=CARTESIAN_POINT ( 'NONE',  ( -6.505213034913026604E-15, 2.500000000000000000, 4.330127018922196314 ) ) ;
#88822=DIRECTION ( 'NONE',  ( 0.000000000000000000, 0.000000000000000000, 1.000000000000000000 ) ) ;
#88823=DIRECTION ( 'NONE',  ( 0.000000000000000000, -0.000000000000000000, 1.000000000000000000 ) ) ;
#88824=AXIS2_PLACEMENT_3D ( 'NONE', #40247, #101092, #120098 ) ;
#88825=CARTESIAN_POINT ( 'NONE',  ( -0.6000000000000323963, 12.50000000000000000, -0.3464101615137759604 ) ) ;
#88826=EDGE_CURVE ( 'NONE', #22678, #111655, #28916, .T. ) ;
#88827=EDGE_LOOP ( 'NONE', ( #72583, #80404, #96969, #126191 ) ) ;
#88828=DIRECTION ( 'NONE',  ( 0.000000000000000000, -0.000000000000000000, 1.000000000000000000 ) ) ;
#88829=VERTEX_POINT ( 'NONE', #17781 ) ;
#88830=DIRECTION ( 'NONE',  ( 0.000000000000000000, 0.000000000000000000, -1.000000000000000000 ) ) ;
#88831=DIRECTION ( 'NONE',  ( -0.000000000000000000, -1.000000000000000000, -0.000000000000000000 ) ) ;
#88832=ADVANCED_FACE ( 'NONE', ( #57731 ), #119880, .T. ) ;
#88833=CARTESIAN_POINT ( 'NONE',  ( 17.17161331427190873, 0.4678040054246561663, 5.513957101009332007 ) ) ;
#88834=DIRECTION ( 'NONE',  ( -0.000000000000000000, 1.000000000000000000, -0.000000000000000000 ) ) ;
#88835=CARTESIAN_POINT ( 'NONE',  ( -3.300000000000027800, 2.500000000000000000, -4.230127018922201998 ) ) ;
#88836=EDGE_CURVE ( 'NONE', #76998, #11828, #109415, .T. ) ;
#88837=ORIENTED_EDGE ( 'NONE', *, *, #19730, .T. ) ;
#88838=AXIS2_PLACEMENT_3D ( 'NONE', #60158, #58847, #51615 ) ;
#88839=EDGE_LOOP ( 'NONE', ( #119235, #79683 ) ) ;
#88840=EDGE_CURVE ( 'NONE', #60021, #46396, #38080, .T. ) ;
#88841=ORIENTED_EDGE ( 'NONE', *, *, #49430, .F. ) ;
#88842=EDGE_LOOP ( 'NONE', ( #96255, #86923 ) ) ;
#88843=VERTEX_POINT ( 'NONE', #38754 ) ;
#88844=DIRECTION ( 'NONE',  ( -0.000000000000000000, -1.000000000000000000, -0.000000000000000000 ) ) ;
#88845=DIRECTION ( 'NONE',  ( -0.000000000000000000, 1.000000000000000000, -0.000000000000000000 ) ) ;
#88846=CIRCLE ( 'NONE', #105578, 0.09999999999999982514 ) ;
#88847=CARTESIAN_POINT ( 'NONE',  ( 2.949999999999946887, 2.500000000000000000, -2.165063509461101710 ) ) ;
#88848=ADVANCED_FACE ( 'NONE', ( #68822 ), #36274, .T. ) ;
#88849=FACE_BOUND ( 'NONE', #117785, .T. ) ;
#88850=CARTESIAN_POINT ( 'NONE',  ( -11.64999999999999680, 2.500000000000000000, 2.857883832488649301 ) ) ;
#88852=CARTESIAN_POINT ( 'NONE',  ( -0.8500000000000382805, 2.500000000000000000, -5.802370205355749988 ) ) ;
#88853=FACE_OUTER_BOUND ( 'NONE', #99209, .T. ) ;
#88854=AXIS2_PLACEMENT_3D ( 'NONE', #77018, #17432, #86832 ) ;
#88855=AXIS2_PLACEMENT_3D ( 'NONE', #13702, #53642, #31435 ) ;
#88856=CIRCLE ( 'NONE', #47013, 0.06509327318403745899 ) ;
#88857=CARTESIAN_POINT ( 'NONE',  ( 2.499999999999947153, 2.500000000000000000, 0.6928203230275494784 ) ) ;
#88859=CARTESIAN_POINT ( 'NONE',  ( -7.900000000000014566, 2.500000000000000000, 0.7928203230275495672 ) ) ;
#88860=DIRECTION ( 'NONE',  ( 0.000000000000000000, 0.000000000000000000, 1.000000000000000000 ) ) ;
#88861=AXIS2_PLACEMENT_3D ( 'NONE', #105039, #33116, #103774 ) ;
#88862=CIRCLE ( 'NONE', #128607, 0.06509327318403745899 ) ;
#88863=CARTESIAN_POINT ( 'NONE',  ( 14.54999999999989235, 2.500000000000000000, -2.165063509461101710 ) ) ;
#88864=ORIENTED_EDGE ( 'NONE', *, *, #85323, .F. ) ;
#88865=ORIENTED_EDGE ( 'NONE', *, *, #102803, .T. ) ;
#88867=ORIENTED_EDGE ( 'NONE', *, *, #81745, .T. ) ;
#88868=CIRCLE ( 'NONE', #57582, 0.1000000000000000472 ) ;
#88869=DIRECTION ( 'NONE',  ( 0.000000000000000000, 0.000000000000000000, 1.000000000000000000 ) ) ;
#88870=CARTESIAN_POINT ( 'NONE',  ( -4.150000000000025224, 12.50000000000000000, 2.857883832488649301 ) ) ;
#88871=FACE_BOUND ( 'NONE', #85872, .T. ) ;
#88872=CARTESIAN_POINT ( 'NONE',  ( -7.900000000000014566, 12.50000000000000000, -5.022947341949754119 ) ) ;
#88873=ORIENTED_EDGE ( 'NONE', *, *, #14597, .T. ) ;
#88874=DIRECTION ( 'NONE',  ( -0.000000000000000000, -1.000000000000000000, -0.000000000000000000 ) ) ;
#88875=CARTESIAN_POINT ( 'NONE',  ( -11.04999999999999893, 2.500000000000000000, 6.048780366869520364 ) ) ;
#88876=DIRECTION ( 'NONE',  ( 0.000000000000000000, -0.9999939076577903929, 0.003490651415223739937 ) ) ;
#88877=CARTESIAN_POINT ( 'NONE',  ( 1.049999999999952971, 12.50000000000000000, 6.148780366869520897 ) ) ;
#88878=DIRECTION ( 'NONE',  ( 0.000000000000000000, 1.000000000000000000, 0.000000000000000000 ) ) ;
#88879=CIRCLE ( 'NONE', #61711, 0.06509327318403745899 ) ;
#88880=ORIENTED_EDGE ( 'NONE', *, *, #119921, .F. ) ;
#88881=CARTESIAN_POINT ( 'NONE',  ( -8.350000000000012079, 2.500000000000000000, -2.957883832488653830 ) ) ;
#88882=ADVANCED_FACE ( 'NONE', ( #110674 ), #35201, .T. ) ;
#88884=VERTEX_POINT ( 'NONE', #123548 ) ;
#88885=EDGE_CURVE ( 'NONE', #23570, #93873, #78122, .T. ) ;
#88886=ORIENTED_EDGE ( 'NONE', *, *, #3691, .T. ) ;
#88887=EDGE_CURVE ( 'NONE', #98236, #21944, #2905, .T. ) ;
#88888=CARTESIAN_POINT ( 'NONE',  ( -4.600000000000028955, 2.500000000000000000, -4.430127018922202176 ) ) ;
#88890=CONICAL_SURFACE ( 'NONE', #107763, 0.09999999999999982514, 0.003490658503988666988 ) ;
#88891=EDGE_CURVE ( 'NONE', #126455, #39511, #57180, .T. ) ;
#88892=ORIENTED_EDGE ( 'NONE', *, *, #59551, .F. ) ;
#88893=AXIS2_PLACEMENT_3D ( 'NONE', #28522, #58636, #88724 ) ;
#88894=EDGE_CURVE ( 'NONE', #65565, #79722, #124075, .T. ) ;
#88895=CIRCLE ( 'NONE', #17870, 0.06509327318403741736 ) ;
#88896=DIRECTION ( 'NONE',  ( 0.000000000000000000, 0.000000000000000000, 1.000000000000000000 ) ) ;
#88897=DIRECTION ( 'NONE',  ( 0.000000000000000000, 0.000000000000000000, -1.000000000000000000 ) ) ;
#88898=ORIENTED_EDGE ( 'NONE', *, *, #13664, .F. ) ;
#88900=EDGE_CURVE ( 'NONE', #105738, #92137, #23748, .T. ) ;
#88901=ORIENTED_EDGE ( 'NONE', *, *, #71151, .F. ) ;
#88902=DIRECTION ( 'NONE',  ( -0.000000000000000000, -1.000000000000000000, -0.000000000000000000 ) ) ;
#88904=CARTESIAN_POINT ( 'NONE',  ( -5.400000000000019895, 12.50000000000000000, -0.7579135962115916003 ) ) ;
#88905=FACE_BOUND ( 'NONE', #58362, .T. ) ;
#88906=EDGE_CURVE ( 'NONE', #33814, #97603, #19526, .T. ) ;
#88907=CIRCLE ( 'NONE', #34552, 0.1000000000000002554 ) ;
#88908=EDGE_CURVE ( 'NONE', #94097, #58339, #84926, .T. ) ;
#88909=ORIENTED_EDGE ( 'NONE', *, *, #10967, .T. ) ;
#88910=VECTOR ( 'NONE', #62013, 1000.000000000000000 ) ;
#88912=EDGE_LOOP ( 'NONE', ( #5660, #101496, #20994, #22076 ) ) ;
#88913=DIRECTION ( 'NONE',  ( 0.000000000000000000, 0.000000000000000000, -1.000000000000000000 ) ) ;
#88914=CARTESIAN_POINT ( 'NONE',  ( -5.850000000000021849, 2.500000000000000000, -2.857883832488653741 ) ) ;
#88915=DIRECTION ( 'NONE',  ( 0.000000000000000000, 0.000000000000000000, 1.000000000000000000 ) ) ;
#88916=CARTESIAN_POINT ( 'NONE',  ( -4.600000000000024514, 12.50000000000000000, 0.7579135962115869374 ) ) ;
#88917=DIRECTION ( 'NONE',  ( -0.000000000000000000, -1.000000000000000000, -0.000000000000000000 ) ) ;
#88918=ORIENTED_EDGE ( 'NONE', *, *, #120326, .T. ) ;
#88919=EDGE_LOOP ( 'NONE', ( #122826, #69037 ) ) ;
#88920=ORIENTED_EDGE ( 'NONE', *, *, #2888, .T. ) ;
#88921=DIRECTION ( 'NONE',  ( 0.000000000000000000, 0.000000000000000000, 1.000000000000000000 ) ) ;
#88922=CIRCLE ( 'NONE', #101439, 0.06509327318403745899 ) ;
#88923=CIRCLE ( 'NONE', #65923, 0.09999999999999982514 ) ;
#88924=DIRECTION ( 'NONE',  ( 0.000000000000000000, -0.000000000000000000, 1.000000000000000000 ) ) ;
#88926=VERTEX_POINT ( 'NONE', #94105 ) ;
#88927=ORIENTED_EDGE ( 'NONE', *, *, #35470, .T. ) ;
#88928=ORIENTED_EDGE ( 'NONE', *, *, #75105, .T. ) ;
#88929=CARTESIAN_POINT ( 'NONE',  ( 5.849999999999933920, 12.50000000000000000, -2.165063509461101710 ) ) ;
#88930=DIRECTION ( 'NONE',  ( -0.000000000000000000, -1.000000000000000000, -0.000000000000000000 ) ) ;
#88932=DIRECTION ( 'NONE',  ( -0.000000000000000000, 1.000000000000000000, -0.000000000000000000 ) ) ;
#88933=CARTESIAN_POINT ( 'NONE',  ( 7.499999999999923617, 12.50000000000000000, 0.6277270498435120194 ) ) ;
#88934=CONICAL_SURFACE ( 'NONE', #42986, 0.1000000000000002554, 0.003490658503988666988 ) ;
#88935=DIRECTION ( 'NONE',  ( 0.000000000000000000, 0.000000000000000000, 1.000000000000000000 ) ) ;
#88936=DIRECTION ( 'NONE',  ( -0.000000000000000000, -1.000000000000000000, -0.000000000000000000 ) ) ;
#88937=CARTESIAN_POINT ( 'NONE',  ( 1.649999999999950617, 12.50000000000000000, 2.165063509461097713 ) ) ;
#88938=AXIS2_PLACEMENT_3D ( 'NONE', #28082, #26789, #47729 ) ;
#88940=VERTEX_POINT ( 'NONE', #24724 ) ;
#88941=ORIENTED_EDGE ( 'NONE', *, *, #12912, .F. ) ;
#88942=CARTESIAN_POINT ( 'NONE',  ( 2.899999999999946620, 2.500000000000000000, -5.022947341949754119 ) ) ;
#88943=VECTOR ( 'NONE', #24082, 1000.000000000000000 ) ;
#88944=AXIS2_PLACEMENT_3D ( 'NONE', #54503, #25690, #55166 ) ;
#88945=CARTESIAN_POINT ( 'NONE',  ( -8.150000000000014566, 2.500000000000000000, -6.048780366869521252 ) ) ;
#88946=ORIENTED_EDGE ( 'NONE', *, *, #50464, .T. ) ;
#88947=EDGE_LOOP ( 'NONE', ( #65075, #45676 ) ) ;
#88948=DIRECTION ( 'NONE',  ( 0.000000000000000000, 0.000000000000000000, 1.000000000000000000 ) ) ;
#88949=CARTESIAN_POINT ( 'NONE',  ( -12.49999999999999289, 12.50000000000000000, 4.957854068765711553 ) ) ;
#88950=CARTESIAN_POINT ( 'NONE',  ( 2.500000000000001776, 2.021986658763282652, -9.892226903609811828 ) ) ;
#88951=AXIS2_PLACEMENT_3D ( 'NONE', #83319, #73472, #102939 ) ;
#88952=CARTESIAN_POINT ( 'NONE',  ( -14.34999999999998543, 2.500000000000000000, -2.511473670974875727 ) ) ;
#88953=EDGE_CURVE ( 'NONE', #88981, #53090, #27939, .T. ) ;
#88954=VECTOR ( 'NONE', #8588, 1000.000000000000000 ) ;
#88955=DIRECTION ( 'NONE',  ( 0.000000000000000000, 0.000000000000000000, 1.000000000000000000 ) ) ;
#88956=FACE_OUTER_BOUND ( 'NONE', #14752, .T. ) ;
#88957=CARTESIAN_POINT ( 'NONE',  ( 10.84999999999990905, 2.500000000000000000, -7.188010851410854052 ) ) ;
#88958=VECTOR ( 'NONE', #55965, 1000.000000000000000 ) ;
#88959=DIRECTION ( 'NONE',  ( -0.000000000000000000, -1.000000000000000000, -0.000000000000000000 ) ) ;
#88960=CIRCLE ( 'NONE', #26174, 0.06509327318403745899 ) ;
#88961=AXIS2_PLACEMENT_3D ( 'NONE', #100956, #11287, #38182 ) ;
#88962=EDGE_LOOP ( 'NONE', ( #117132, #95289 ) ) ;
#88963=VECTOR ( 'NONE', #37573, 1000.000000000000000 ) ;
#88964=ORIENTED_EDGE ( 'NONE', *, *, #107949, .F. ) ;
#88965=CONICAL_SURFACE ( 'NONE', #32551, 0.1000000000000002554, 0.003490658503988666988 ) ;
#88967=VERTEX_POINT ( 'NONE', #54190 ) ;
#88968=LINE ( 'NONE', #69976, #62928 ) ;
#88969=CARTESIAN_POINT ( 'NONE',  ( -1.850000000000033840, 2.500000000000000000, 1.918653347947321564 ) ) ;
#88972=CARTESIAN_POINT ( 'NONE',  ( 17.50000000000000000, -0.9166666666666678509, -9.999999999999998224 ) ) ;
#88973=CARTESIAN_POINT ( 'NONE',  ( -8.750000000000008882, 2.500000000000000000, 1.472243186433545459 ) ) ;
#88974=DIRECTION ( 'NONE',  ( 0.000000000000000000, 0.000000000000000000, 1.000000000000000000 ) ) ;
#88975=ORIENTED_EDGE ( 'NONE', *, *, #36256, .T. ) ;
#88976=CARTESIAN_POINT ( 'NONE',  ( -10.00000000000000533, 12.50000000000000000, 5.022947341949748790 ) ) ;
#88977=CIRCLE ( 'NONE', #30415, 0.06509327318403745899 ) ;
#88978=CARTESIAN_POINT ( 'NONE',  ( 7.699999999999923794, 2.500000000000000000, 4.576537180435972019 ) ) ;
#88979=VERTEX_POINT ( 'NONE', #3159 ) ;
#88980=ORIENTED_EDGE ( 'NONE', *, *, #113153, .T. ) ;
#88981=VERTEX_POINT ( 'NONE', #63359 ) ;
#88982=EDGE_LOOP ( 'NONE', ( #72786, #50925 ) ) ;
#88983=DIRECTION ( 'NONE',  ( 0.000000000000000000, 0.000000000000000000, 1.000000000000000000 ) ) ;
#88984=AXIS2_PLACEMENT_3D ( 'NONE', #79247, #119154, #57670 ) ;
#88985=AXIS2_PLACEMENT_3D ( 'NONE', #88564, #99040, #48655 ) ;
#88986=CARTESIAN_POINT ( 'NONE',  ( -14.34999999999998543, 12.50000000000000000, -2.576566944158912964 ) ) ;
#88987=DIRECTION ( 'NONE',  ( 0.000000000000000000, 0.000000000000000000, 1.000000000000000000 ) ) ;
#88988=VECTOR ( 'NONE', #72302, 1000.000000000000000 ) ;
#88989=EDGE_CURVE ( 'NONE', #46456, #107304, #99046, .T. ) ;
#88990=CIRCLE ( 'NONE', #43317, 0.06509327318403745899 ) ;
#88991=VERTEX_POINT ( 'NONE', #25345 ) ;
#88992=CARTESIAN_POINT ( 'NONE',  ( 5.399999999999936406, 2.500000000000000000, -3.637306695894650055 ) ) ;
#88993=DIRECTION ( 'NONE',  ( -0.000000000000000000, 1.000000000000000000, -0.000000000000000000 ) ) ;
#88994=ADVANCED_FACE ( 'NONE', ( #73179 ), #34565, .T. ) ;
#88995=DIRECTION ( 'NONE',  ( 0.000000000000000000, 0.000000000000000000, 1.000000000000000000 ) ) ;
#88996=CARTESIAN_POINT ( 'NONE',  ( -0.4000000000000404898, 12.50000000000000000, 5.022947341949748790 ) ) ;
#88997=EDGE_CURVE ( 'NONE', #9756, #30789, #53546, .T. ) ;
#88998=CONICAL_SURFACE ( 'NONE', #78551, 0.1000000000000000056, 0.003490658503988666988 ) ;
#88999=EDGE_LOOP ( 'NONE', ( #74076, #31600 ) ) ;
#89000=DIRECTION ( 'NONE',  ( -4.274815082592931898E-19, -0.9999939076577903929, -0.003490651415223739937 ) ) ;
#89001=AXIS2_PLACEMENT_3D ( 'NONE', #14358, #123050, #84401 ) ;
#89002=AXIS2_PLACEMENT_3D ( 'NONE', #4335, #55405, #93397 ) ;
#89003=EDGE_LOOP ( 'NONE', ( #128688, #29663, #34572, #23878 ) ) ;
#89004=EDGE_CURVE ( 'NONE', #6453, #86025, #115013, .T. ) ;
#89005=EDGE_CURVE ( 'NONE', #5867, #121928, #94837, .T. ) ;
#89006=ORIENTED_EDGE ( 'NONE', *, *, #14565, .F. ) ;
#89007=DIRECTION ( 'NONE',  ( 0.000000000000000000, 1.000000000000000000, 0.000000000000000000 ) ) ;
#89008=ADVANCED_FACE ( 'NONE', ( #84277 ), #34220, .T. ) ;
#89009=FACE_OUTER_BOUND ( 'NONE', #116630, .T. ) ;
#89010=ADVANCED_FACE ( 'NONE', ( #54809 ), #23409, .T. ) ;
#89011=FACE_BOUND ( 'NONE', #97153, .T. ) ;
#89012=CARTESIAN_POINT ( 'NONE',  ( -11.24999999999996447, 2.500000000000000000, -6.495190528383298911 ) ) ;
#89013=DIRECTION ( 'NONE',  ( 0.000000000000000000, 0.000000000000000000, -1.000000000000000000 ) ) ;
#89014=DIRECTION ( 'NONE',  ( -4.274815082592931898E-19, -0.9999939076577903929, -0.003490651415223739937 ) ) ;
#89015=VECTOR ( 'NONE', #36879, 1000.000000000000000 ) ;
#89016=AXIS2_PLACEMENT_3D ( 'NONE', #33532, #25613, #115938 ) ;
#89017=ORIENTED_EDGE ( 'NONE', *, *, #18254, .T. ) ;
#89018=DIRECTION ( 'NONE',  ( -0.000000000000000000, 1.000000000000000000, -0.000000000000000000 ) ) ;
#89019=DIRECTION ( 'NONE',  ( 0.000000000000000000, -0.9999939076577903929, 0.003490651415223739937 ) ) ;
#89021=LINE ( 'NONE', #98824, #17406 ) ;
#89022=CARTESIAN_POINT ( 'NONE',  ( -0.8500000000000382805, 12.50000000000000000, -1.472243186433550122 ) ) ;
#89023=ORIENTED_EDGE ( 'NONE', *, *, #118434, .F. ) ;
#89024=PLANE ( 'NONE',  #120131 ) ;
#89025=FACE_OUTER_BOUND ( 'NONE', #70032, .T. ) ;
#89026=ORIENTED_EDGE ( 'NONE', *, *, #6829, .T. ) ;
#89027=EDGE_LOOP ( 'NONE', ( #64168, #45944 ) ) ;
#89028=FACE_OUTER_BOUND ( 'NONE', #48045, .T. ) ;
#89029=LINE ( 'NONE', #121058, #38110 ) ;
#89030=FACE_BOUND ( 'NONE', #82834, .T. ) ;
#89031=CARTESIAN_POINT ( 'NONE',  ( 15.40649769635636801, -2.500000000000000000, -5.817321165395405558 ) ) ;
#89032=AXIS2_PLACEMENT_3D ( 'NONE', #97101, #108199, #26437 ) ;
#89033=DIRECTION ( 'NONE',  ( 0.000000000000000000, 0.000000000000000000, 1.000000000000000000 ) ) ;
#89034=CIRCLE ( 'NONE', #74457, 0.1000000000000002554 ) ;
#89035=ORIENTED_EDGE ( 'NONE', *, *, #81354, .F. ) ;
#89036=LINE ( 'NONE', #128333, #128207 ) ;
#89037=ADVANCED_FACE ( 'NONE', ( #58693 ), #7643, .T. ) ;
#89039=ORIENTED_EDGE ( 'NONE', *, *, #121583, .F. ) ;
#89040=DIRECTION ( 'NONE',  ( 0.000000000000000000, 0.000000000000000000, 1.000000000000000000 ) ) ;
#89041=DIRECTION ( 'NONE',  ( 0.000000000000000000, 0.000000000000000000, 1.000000000000000000 ) ) ;
#89042=AXIS2_PLACEMENT_3D ( 'NONE', #98459, #11383, #68369 ) ;
#89043=ADVANCED_FACE ( 'NONE', ( #75741 ), #115664, .T. ) ;
#89044=FACE_OUTER_BOUND ( 'NONE', #37493, .T. ) ;
#89045=FACE_OUTER_BOUND ( 'NONE', #680, .T. ) ;
#89046=ADVANCED_FACE ( 'NONE', ( #126794 ), #67635, .T. ) ;
#89047=ORIENTED_EDGE ( 'NONE', *, *, #35213, .T. ) ;
#89048=EDGE_CURVE ( 'NONE', #27272, #21509, #107792, .T. ) ;
#89049=VECTOR ( 'NONE', #39997, 1000.000000000000000 ) ;
#89050=DIRECTION ( 'NONE',  ( -0.000000000000000000, -1.000000000000000000, -0.000000000000000000 ) ) ;
#89051=PLANE ( 'NONE',  #33098 ) ;
#89052=DIRECTION ( 'NONE',  ( 0.000000000000000000, 1.000000000000000000, 0.000000000000000000 ) ) ;
#89053=AXIS2_PLACEMENT_3D ( 'NONE', #1230, #102014, #29415 ) ;
#89054=CARTESIAN_POINT ( 'NONE',  ( 16.56034314470449686, -0.8287381876616503051, -6.090234461610894101 ) ) ;
#89055=ORIENTED_EDGE ( 'NONE', *, *, #52677, .F. ) ;
#89056=EDGE_LOOP ( 'NONE', ( #57100, #104713 ) ) ;
#89057=EDGE_CURVE ( 'NONE', #80664, #71349, #65589, .T. ) ;
#89058=CARTESIAN_POINT ( 'NONE',  ( 16.98713617295328149, 1.503435538382916326, 5.629434171173037349 ) ) ;
#89059=EDGE_CURVE ( 'NONE', #95554, #34514, #46955, .T. ) ;
#89060=ORIENTED_EDGE ( 'NONE', *, *, #45118, .T. ) ;
#89061=CARTESIAN_POINT ( 'NONE',  ( 8.099999999999921485, 12.50000000000000000, -0.3464101615137783474 ) ) ;
#89062=FACE_OUTER_BOUND ( 'NONE', #121492, .T. ) ;
#89063=EDGE_CURVE ( 'NONE', #80857, #95501, #63449, .T. ) ;
#89064=DIRECTION ( 'NONE',  ( 0.000000000000000000, -0.000000000000000000, 1.000000000000000000 ) ) ;
#89065=ADVANCED_FACE ( 'NONE', ( #77045 ), #118253, .T. ) ;
#89066=CARTESIAN_POINT ( 'NONE',  ( -13.94999999999998863, 12.50000000000000000, -1.818653347947323917 ) ) ;
#89067=ORIENTED_EDGE ( 'NONE', *, *, #80606, .F. ) ;
#89068=CARTESIAN_POINT ( 'NONE',  ( -13.74999999999998934, 12.50000000000000000, -1.537336459617585360 ) ) ;
#89069=DIRECTION ( 'NONE',  ( -4.274815082592931898E-19, -0.9999939076577903929, -0.003490651415223739937 ) ) ;
#89070=CARTESIAN_POINT ( 'NONE',  ( -3.150000000000032330, 2.500000000000000000, -6.048780366869526581 ) ) ;
#89072=FACE_OUTER_BOUND ( 'NONE', #19947, .T. ) ;
#89074=DIRECTION ( 'NONE',  ( 0.000000000000000000, 1.000000000000000000, 0.000000000000000000 ) ) ;
#89075=EDGE_CURVE ( 'NONE', #53805, #31468, #9157, .T. ) ;
#89076=EDGE_LOOP ( 'NONE', ( #79089, #120369 ) ) ;
#89077=ORIENTED_EDGE ( 'NONE', *, *, #6742, .T. ) ;
#89078=CARTESIAN_POINT ( 'NONE',  ( 3.349999999999945466, 12.50000000000000000, -6.495190528383302464 ) ) ;
#89079=ORIENTED_EDGE ( 'NONE', *, *, #64153, .T. ) ;
#89080=FACE_OUTER_BOUND ( 'NONE', #82165, .T. ) ;
#89081=ORIENTED_EDGE ( 'NONE', *, *, #107477, .F. ) ;
#89083=ORIENTED_EDGE ( 'NONE', *, *, #29198, .F. ) ;
#89084=PLANE ( 'NONE',  #37458 ) ;
#89085=AXIS2_PLACEMENT_3D ( 'NONE', #15269, #125251, #95150 ) ;
#89087=DIRECTION ( 'NONE',  ( -0.000000000000000000, -1.000000000000000000, -0.000000000000000000 ) ) ;
#89088=DIRECTION ( 'NONE',  ( 0.000000000000000000, 1.000000000000000000, 0.000000000000000000 ) ) ;
#89089=CIRCLE ( 'NONE', #39033, 0.06509327318403745899 ) ;
#89090=FACE_OUTER_BOUND ( 'NONE', #40268, .T. ) ;
#89091=DIRECTION ( 'NONE',  ( 0.000000000000000000, 0.000000000000000000, 1.000000000000000000 ) ) ;
#89092=FACE_OUTER_BOUND ( 'NONE', #4850, .T. ) ;
#89093=CARTESIAN_POINT ( 'NONE',  ( 13.74999999999989697, 2.500000000000000000, 2.757883832488649656 ) ) ;
#89094=DIRECTION ( 'NONE',  ( 0.000000000000000000, 0.000000000000000000, -1.000000000000000000 ) ) ;
#89095=ORIENTED_EDGE ( 'NONE', *, *, #83856, .F. ) ;
#89096=AXIS2_PLACEMENT_3D ( 'NONE', #86253, #36550, #26712 ) ;
#89097=ORIENTED_EDGE ( 'NONE', *, *, #31540, .F. ) ;
#89098=CIRCLE ( 'NONE', #116266, 0.1000000000000002554 ) ;
#89099=AXIS2_PLACEMENT_3D ( 'NONE', #118186, #16735, #96592 ) ;
#89100=DIRECTION ( 'NONE',  ( 0.000000000000000000, 0.000000000000000000, 1.000000000000000000 ) ) ;
#89101=VERTEX_POINT ( 'NONE', #18112 ) ;
#89102=VERTEX_POINT ( 'NONE', #128081 ) ;
#89103=CARTESIAN_POINT ( 'NONE',  ( 6.649999999999928413, 12.50000000000000000, 1.537336459617582918 ) ) ;
#89104=CARTESIAN_POINT ( 'NONE',  ( -5.850000000000021849, 12.50000000000000000, -5.867463478539787225 ) ) ;
#89105=EDGE_CURVE ( 'NONE', #53017, #117711, #116948, .T. ) ;
#89106=CARTESIAN_POINT ( 'NONE',  ( -13.74999999999995381, 2.500000000000000000, 2.265063509461101354 ) ) ;
#89107=DIRECTION ( 'NONE',  ( 0.000000000000000000, 0.000000000000000000, 1.000000000000000000 ) ) ;
#89108=CARTESIAN_POINT ( 'NONE',  ( 12.49999999999990408, 12.50000000000000000, 5.022947341949748790 ) ) ;
#89109=ORIENTED_EDGE ( 'NONE', *, *, #43106, .F. ) ;
#89110=EDGE_LOOP ( 'NONE', ( #127997, #114155, #40773, #98328 ) ) ;
#89111=DIRECTION ( 'NONE',  ( 0.000000000000000000, 0.000000000000000000, 1.000000000000000000 ) ) ;
#89112=EDGE_LOOP ( 'NONE', ( #56363, #58742, #112417, #85982 ) ) ;
#89113=DIRECTION ( 'NONE',  ( 0.000000000000000000, 0.000000000000000000, 1.000000000000000000 ) ) ;
#89114=ORIENTED_EDGE ( 'NONE', *, *, #125996, .F. ) ;
#89115=EDGE_CURVE ( 'NONE', #110068, #47774, #42633, .T. ) ;
#89116=EDGE_LOOP ( 'NONE', ( #9448, #126363, #7178, #44458 ) ) ;
#89117=DIRECTION ( 'NONE',  ( -0.000000000000000000, -1.000000000000000000, -0.000000000000000000 ) ) ;
#89118=DIRECTION ( 'NONE',  ( 0.000000000000000000, 0.000000000000000000, 1.000000000000000000 ) ) ;
#89119=AXIS2_PLACEMENT_3D ( 'NONE', #5977, #13221, #114651 ) ;
#89120=CARTESIAN_POINT ( 'NONE',  ( -13.74999999999995381, 2.500000000000000000, 2.165063509461101265 ) ) ;
#89121=CONICAL_SURFACE ( 'NONE', #34861, 0.1000000000000002554, 0.003490658503988666988 ) ;
#89122=CARTESIAN_POINT ( 'NONE',  ( -7.300000000000013145, 12.50000000000000000, 4.048810130592458201 ) ) ;
#89123=LINE ( 'NONE', #67523, #86808 ) ;
#89124=ORIENTED_EDGE ( 'NONE', *, *, #79295, .F. ) ;
#89125=LINE ( 'NONE', #17121, #125107 ) ;
#89126=DIRECTION ( 'NONE',  ( -4.274815082592931898E-19, -0.9999939076577903929, -0.003490651415223739937 ) ) ;
#89127=FACE_OUTER_BOUND ( 'NONE', #1799, .T. ) ;
#89128=DIRECTION ( 'NONE',  ( 0.000000000000000000, 0.000000000000000000, 1.000000000000000000 ) ) ;
#89129=CIRCLE ( 'NONE', #32720, 0.1000000000000002554 ) ;
#89130=CONICAL_SURFACE ( 'NONE', #9712, 0.1000000000000002554, 0.003490658503988666988 ) ;
#89131=DIRECTION ( 'NONE',  ( 0.000000000000000000, 1.000000000000000000, 0.000000000000000000 ) ) ;
#89132=VERTEX_POINT ( 'NONE', #96038 ) ;
#89133=ORIENTED_EDGE ( 'NONE', *, *, #98916, .F. ) ;
#89134=CARTESIAN_POINT ( 'NONE',  ( -3.150000000000029665, 12.50000000000000000, 6.776507416713035248 ) ) ;
#89135=ORIENTED_EDGE ( 'NONE', *, *, #63929, .F. ) ;
#89136=AXIS2_PLACEMENT_3D ( 'NONE', #43430, #34894, #123880 ) ;
#89137=DIRECTION ( 'NONE',  ( -0.000000000000000000, -1.000000000000000000, -0.000000000000000000 ) ) ;
#89138=CARTESIAN_POINT ( 'NONE',  ( 0.4499999999999573785, 2.500000000000000000, -6.595190528383302109 ) ) ;
#89139=ADVANCED_FACE ( 'NONE', ( #88115 ), #46820, .T. ) ;
#89140=ORIENTED_EDGE ( 'NONE', *, *, #114309, .T. ) ;
#89141=DIRECTION ( 'NONE',  ( 0.000000000000000000, 1.000000000000000000, 0.000000000000000000 ) ) ;
#89142=CARTESIAN_POINT ( 'NONE',  ( -0.4000000000000339950, 2.500000000000000000, 0.6928203230275518099 ) ) ;
#89143=DIRECTION ( 'NONE',  ( 0.000000000000000000, 1.000000000000000000, 0.000000000000000000 ) ) ;
#89144=LINE ( 'NONE', #37488, #124995 ) ;
#89145=VERTEX_POINT ( 'NONE', #56100 ) ;
#89146=EDGE_CURVE ( 'NONE', #117684, #102868, #9254, .T. ) ;
#89147=DIRECTION ( 'NONE',  ( -4.274815082592931898E-19, -0.9999939076577903929, -0.003490651415223739937 ) ) ;
#89148=ORIENTED_EDGE ( 'NONE', *, *, #18236, .T. ) ;
#89149=ADVANCED_FACE ( 'NONE', ( #36497 ), #113717, .T. ) ;
#89150=EDGE_CURVE ( 'NONE', #114153, #104101, #99142, .T. ) ;
#89151=EDGE_CURVE ( 'NONE', #105503, #111361, #21787, .T. ) ;
#89152=CARTESIAN_POINT ( 'NONE',  ( 32.27132508960535517, 3.178320084206410545, -3.140934779234540564 ) ) ;
#89153=EDGE_CURVE ( 'NONE', #84568, #29080, #20069, .T. ) ;
#89154=AXIS2_PLACEMENT_3D ( 'NONE', #497, #8387, #107882 ) ;
#89155=EDGE_CURVE ( 'NONE', #22461, #70010, #28035, .T. ) ;
#89157=CARTESIAN_POINT ( 'NONE',  ( -4.350000000000027178, 2.500000000000000000, -6.841600689897077814 ) ) ;
#89159=AXIS2_PLACEMENT_3D ( 'NONE', #44233, #44901, #105747 ) ;
#89160=DIRECTION ( 'NONE',  ( 0.000000000000000000, 0.000000000000000000, -1.000000000000000000 ) ) ;
#89161=AXIS2_PLACEMENT_3D ( 'NONE', #19507, #30640, #120299 ) ;
#89162=EDGE_LOOP ( 'NONE', ( #112892, #68605, #99756, #127229 ) ) ;
#89163=CARTESIAN_POINT ( 'NONE',  ( -11.25000000000000178, 2.500000000000000000, -5.702370205355745902 ) ) ;
#89164=DIRECTION ( 'NONE',  ( 0.000000000000000000, 0.000000000000000000, -1.000000000000000000 ) ) ;
#89165=ADVANCED_FACE ( 'NONE', ( #61929 ), #109509, .T. ) ;
#89166=DIRECTION ( 'NONE',  ( 0.000000000000000000, 0.000000000000000000, 1.000000000000000000 ) ) ;
#89167=AXIS2_PLACEMENT_3D ( 'NONE', #808, #100932, #40767 ) ;
#89168=VERTEX_POINT ( 'NONE', #99274 ) ;
#89169=ADVANCED_FACE ( 'NONE', ( #31816 ), #109052, .T. ) ;
#89170=DIRECTION ( 'NONE',  ( -0.000000000000000000, 1.000000000000000000, -0.000000000000000000 ) ) ;
#89171=EDGE_CURVE ( 'NONE', #41154, #64623, #115852, .T. ) ;
#89172=VECTOR ( 'NONE', #105294, 1000.000000000000000 ) ;
#89173=CARTESIAN_POINT ( 'NONE',  ( 9.349999999999916156, 2.500000000000000000, -2.611473670974877592 ) ) ;
#89174=EDGE_LOOP ( 'NONE', ( #100342, #81296 ) ) ;
#89175=CARTESIAN_POINT ( 'NONE',  ( 2.899999999999946620, 12.50000000000000000, -3.702399969078687292 ) ) ;
#89176=EDGE_LOOP ( 'NONE', ( #63666, #9497, #55048, #93378 ) ) ;
#89177=DIRECTION ( 'NONE',  ( -4.274815082592931898E-19, -0.9999939076577903929, -0.003490651415223739937 ) ) ;
#89178=VECTOR ( 'NONE', #124596, 1000.000000000000000 ) ;
#89179=VECTOR ( 'NONE', #71868, 1000.000000000000000 ) ;
#89180=CONICAL_SURFACE ( 'NONE', #112174, 0.09999999999999982514, 0.003490658503988666988 ) ;
#89181=ORIENTED_EDGE ( 'NONE', *, *, #5843, .F. ) ;
#89182=CARTESIAN_POINT ( 'NONE',  ( -1.250000000000037970, 12.50000000000000000, 7.122917578226811486 ) ) ;
#89183=CARTESIAN_POINT ( 'NONE',  ( -1.850000000000033840, 2.500000000000000000, 6.248780366869521430 ) ) ;
#89184=ORIENTED_EDGE ( 'NONE', *, *, #101850, .T. ) ;
#89185=ORIENTED_EDGE ( 'NONE', *, *, #107782, .T. ) ;
#89186=CARTESIAN_POINT ( 'NONE',  ( -10.85000000000000142, 2.500000000000000000, -1.572243186433546214 ) ) ;
#89187=FACE_OUTER_BOUND ( 'NONE', #83545, .T. ) ;
#89188=ORIENTED_EDGE ( 'NONE', *, *, #88725, .F. ) ;
#89189=CARTESIAN_POINT ( 'NONE',  ( 8.299999999999922551, 12.50000000000000000, -4.330127018922201643 ) ) ;
#89190=DIRECTION ( 'NONE',  ( 0.000000000000000000, 1.000000000000000000, 0.000000000000000000 ) ) ;
#89191=DIRECTION ( 'NONE',  ( -0.000000000000000000, -1.000000000000000000, -0.000000000000000000 ) ) ;
#89193=CARTESIAN_POINT ( 'NONE',  ( -11.25000000000000178, 2.500000000000000000, -5.802370205355746435 ) ) ;
#89194=CARTESIAN_POINT ( 'NONE',  ( -9.600000000000008527, 2.500000000000000000, -2.385244779468109755E-15 ) ) ;
#89195=LINE ( 'NONE', #150, #71358 ) ;
#89196=ORIENTED_EDGE ( 'NONE', *, *, #125777, .F. ) ;
#89197=ORIENTED_EDGE ( 'NONE', *, *, #20289, .F. ) ;
#89198=EDGE_LOOP ( 'NONE', ( #104024, #104512 ) ) ;
#89199=ORIENTED_EDGE ( 'NONE', *, *, #62771, .F. ) ;
#89200=CARTESIAN_POINT ( 'NONE',  ( -10.20000000000000639, 2.500000000000000000, -3.983716857408421852 ) ) ;
#89201=DIRECTION ( 'NONE',  ( 1.000000000000000000, 0.000000000000000000, 0.000000000000000000 ) ) ;
#89202=CARTESIAN_POINT ( 'NONE',  ( -1.450000000000035927, 2.500000000000000000, -1.718653347947326049 ) ) ;
#89204=FACE_BOUND ( 'NONE', #28146, .T. ) ;
#89205=VERTEX_POINT ( 'NONE', #50812 ) ;
#89206=EDGE_CURVE ( 'NONE', #48509, #90525, #78217, .T. ) ;
#89207=CARTESIAN_POINT ( 'NONE',  ( 12.49999999999990585, 2.500000000000000000, 3.737306695894644371 ) ) ;
#89208=DIRECTION ( 'NONE',  ( -4.274815082592931898E-19, -0.9999939076577903929, -0.003490651415223739937 ) ) ;
#89209=EDGE_CURVE ( 'NONE', #32144, #40462, #3000, .T. ) ;
#89211=AXIS2_PLACEMENT_3D ( 'NONE', #33388, #32746, #73283 ) ;
#89212=DIRECTION ( 'NONE',  ( -0.000000000000000000, 1.000000000000000000, -0.000000000000000000 ) ) ;
#89213=AXIS2_PLACEMENT_3D ( 'NONE', #85098, #23605, #104725 ) ;
#89214=ADVANCED_FACE ( 'NONE', ( #88796 ), #129397, .T. ) ;
#89215=LINE ( 'NONE', #129170, #38181 ) ;
#89216=CARTESIAN_POINT ( 'NONE',  ( -7.700000000000014388, 2.500000000000000000, -4.676537180435977881 ) ) ;
#89217=CARTESIAN_POINT ( 'NONE',  ( 10.84999999999991260, 12.50000000000000000, 6.430097255199259010 ) ) ;
#89218=DIRECTION ( 'NONE',  ( 0.000000000000000000, 0.000000000000000000, 1.000000000000000000 ) ) ;
#89219=CARTESIAN_POINT ( 'NONE',  ( -4.150000000000027889, 2.500000000000000000, -6.595190528383302109 ) ) ;
#89220=CARTESIAN_POINT ( 'NONE',  ( -6.050000000000017586, 2.500000000000000000, 1.718653347947321386 ) ) ;
#89221=ADVANCED_FACE ( 'NONE', ( #128752 ), #36463, .T. ) ;
#89222=CIRCLE ( 'NONE', #34953, 0.06509327318403745899 ) ;
#89224=ORIENTED_EDGE ( 'NONE', *, *, #122745, .F. ) ;
#89226=EDGE_LOOP ( 'NONE', ( #17395, #63621, #59623, #23290 ) ) ;
#89227=CARTESIAN_POINT ( 'NONE',  ( 17.28959186693577266, -1.567451025696849021, -5.035561754033041737 ) ) ;
#89228=DIRECTION ( 'NONE',  ( 0.000000000000000000, 1.000000000000000000, 0.000000000000000000 ) ) ;
#89229=ORIENTED_EDGE ( 'NONE', *, *, #77801, .F. ) ;
#89230=ORIENTED_EDGE ( 'NONE', *, *, #61890, .F. ) ;
#89231=VECTOR ( 'NONE', #95662, 1000.000000000000000 ) ;
#89232=ORIENTED_EDGE ( 'NONE', *, *, #70586, .T. ) ;
#89233=DIRECTION ( 'NONE',  ( -0.000000000000000000, -1.000000000000000000, -0.000000000000000000 ) ) ;
#89235=DIRECTION ( 'NONE',  ( 0.000000000000000000, 0.000000000000000000, 1.000000000000000000 ) ) ;
#89236=CARTESIAN_POINT ( 'NONE',  ( -5.200000000000022382, 2.500000000000000000, 0.2464101615137735679 ) ) ;
#89237=DIRECTION ( 'NONE',  ( 0.000000000000000000, -0.9999939076577903929, 0.003490651415223739937 ) ) ;
#89238=CARTESIAN_POINT ( 'NONE',  ( 10.39999999999991154, 2.500000000000000000, -3.637306695894650055 ) ) ;
#89240=DIRECTION ( 'NONE',  ( -0.000000000000000000, 1.000000000000000000, -0.000000000000000000 ) ) ;
#89241=EDGE_CURVE ( 'NONE', #118034, #11372, #65673, .T. ) ;
#89242=VERTEX_POINT ( 'NONE', #69802 ) ;
#89243=DIRECTION ( 'NONE',  ( -0.000000000000000000, -1.000000000000000000, -0.000000000000000000 ) ) ;
#89244=ORIENTED_EDGE ( 'NONE', *, *, #62731, .F. ) ;
#89245=VERTEX_POINT ( 'NONE', #51465 ) ;
#89246=VERTEX_POINT ( 'NONE', #40357 ) ;
#89247=CARTESIAN_POINT ( 'NONE',  ( 4.799999999999934097, 12.50000000000000000, 4.676537180435972552 ) ) ;
#89248=EDGE_LOOP ( 'NONE', ( #125259, #2600 ) ) ;
#89249=AXIS2_PLACEMENT_3D ( 'NONE', #50127, #78298, #28540 ) ;
#89250=VERTEX_POINT ( 'NONE', #1691 ) ;
#89251=AXIS2_PLACEMENT_3D ( 'NONE', #122399, #73279, #34009 ) ;
#89252=CIRCLE ( 'NONE', #5603, 0.1000000000000002554 ) ;
#89253=CARTESIAN_POINT ( 'NONE',  ( 10.84999999999990905, 2.500000000000000000, 1.572243186433545548 ) ) ;
#89254=DIRECTION ( 'NONE',  ( -0.000000000000000000, 1.000000000000000000, -0.000000000000000000 ) ) ;
#89255=DIRECTION ( 'NONE',  ( 0.000000000000000000, 1.000000000000000000, 0.000000000000000000 ) ) ;
#89256=CIRCLE ( 'NONE', #80945, 0.09999999999999999167 ) ;
#89257=EDGE_CURVE ( 'NONE', #78294, #3186, #7078, .T. ) ;
#89258=CARTESIAN_POINT ( 'NONE',  ( -13.54999999999999005, 12.50000000000000000, 2.511473670974877503 ) ) ;
#89259=FACE_OUTER_BOUND ( 'NONE', #5560, .T. ) ;
#89260=CONICAL_SURFACE ( 'NONE', #76647, 0.1000000000000002554, 0.003490658503988666988 ) ;
#89261=VERTEX_POINT ( 'NONE', #109730 ) ;
#89262=DIRECTION ( 'NONE',  ( -4.274815082592931898E-19, -0.9999939076577903929, -0.003490651415223739937 ) ) ;
#89263=AXIS2_PLACEMENT_3D ( 'NONE', #15110, #5310, #95002 ) ;
#89264=ORIENTED_EDGE ( 'NONE', *, *, #22588, .F. ) ;
#89265=VECTOR ( 'NONE', #36835, 1000.000000000000000 ) ;
#89266=DIRECTION ( 'NONE',  ( -4.274815082592931898E-19, -0.9999939076577903929, -0.003490651415223739937 ) ) ;
#89267=ORIENTED_EDGE ( 'NONE', *, *, #40416, .T. ) ;
#89268=DIRECTION ( 'NONE',  ( -0.000000000000000000, 1.000000000000000000, -0.000000000000000000 ) ) ;
#89269=CARTESIAN_POINT ( 'NONE',  ( 8.749999999999921840, 12.50000000000000000, 2.857883832488649301 ) ) ;
#89270=ORIENTED_EDGE ( 'NONE', *, *, #68797, .F. ) ;
#89271=DIRECTION ( 'NONE',  ( 0.000000000000000000, 0.000000000000000000, 1.000000000000000000 ) ) ;
#89272=AXIS2_PLACEMENT_3D ( 'NONE', #124977, #45783, #56851 ) ;
#89273=EDGE_CURVE ( 'NONE', #118968, #27375, #13348, .T. ) ;
#89274=DIRECTION ( 'NONE',  ( 0.000000000000000000, 1.000000000000000000, 0.000000000000000000 ) ) ;
#89275=EDGE_LOOP ( 'NONE', ( #126914, #15381, #88150, #53533 ) ) ;
#89276=AXIS2_PLACEMENT_3D ( 'NONE', #38824, #116691, #117982 ) ;
#89277=CIRCLE ( 'NONE', #80878, 0.09999999999999982514 ) ;
#89278=AXIS2_PLACEMENT_3D ( 'NONE', #56207, #34671, #5170 ) ;
#89279=DIRECTION ( 'NONE',  ( 0.000000000000000000, 0.000000000000000000, -1.000000000000000000 ) ) ;
#89280=VERTEX_POINT ( 'NONE', #71737 ) ;
#89281=ADVANCED_FACE ( 'NONE', ( #111666 ), #48890, .T. ) ;
#89282=VERTEX_POINT ( 'NONE', #122138 ) ;
#89283=DIRECTION ( 'NONE',  ( 0.000000000000000000, 0.000000000000000000, 1.000000000000000000 ) ) ;
#89284=DIRECTION ( 'NONE',  ( 0.000000000000000000, 0.000000000000000000, 1.000000000000000000 ) ) ;
#89286=DIRECTION ( 'NONE',  ( 0.000000000000000000, -0.9999939076577903929, 0.003490651415223739937 ) ) ;
#89287=DIRECTION ( 'NONE',  ( -4.274815082592931898E-19, -0.9999939076577903929, -0.003490651415223739937 ) ) ;
#89288=VERTEX_POINT ( 'NONE', #34411 ) ;
#89290=CIRCLE ( 'NONE', #32876, 0.1000000000000000472 ) ;
#89291=ORIENTED_EDGE ( 'NONE', *, *, #90194, .T. ) ;
#89292=LINE ( 'NONE', #59209, #125898 ) ;
#89293=CARTESIAN_POINT ( 'NONE',  ( -11.25000000000000000, 2.500000000000000000, -2.857883832488649745 ) ) ;
#89294=ADVANCED_FACE ( 'NONE', ( #93956 ), #40582, .T. ) ;
#89296=DIRECTION ( 'NONE',  ( -0.000000000000000000, 1.000000000000000000, -0.000000000000000000 ) ) ;
#89297=CARTESIAN_POINT ( 'NONE',  ( -4.150000000000025224, 12.50000000000000000, 6.495190528383297135 ) ) ;
#89299=DIRECTION ( 'NONE',  ( 0.000000000000000000, 0.000000000000000000, 1.000000000000000000 ) ) ;
#89300=VERTEX_POINT ( 'NONE', #3001 ) ;
#89302=CIRCLE ( 'NONE', #49614, 0.06509327318403745899 ) ;
#89303=CARTESIAN_POINT ( 'NONE',  ( 4.199999999999939782, 12.50000000000000000, 0.06509327318403515528 ) ) ;
#89304=AXIS2_PLACEMENT_3D ( 'NONE', #20883, #60805, #11041 ) ;
#89305=DIRECTION ( 'NONE',  ( -0.000000000000000000, -1.000000000000000000, -0.000000000000000000 ) ) ;
#89306=EDGE_CURVE ( 'NONE', #100844, #128715, #70687, .T. ) ;
#89307=EDGE_CURVE ( 'NONE', #51386, #43124, #14082, .T. ) ;
#89308=EDGE_CURVE ( 'NONE', #74070, #59844, #119975, .T. ) ;
#89309=ADVANCED_FACE ( 'NONE', ( #33120 ), #30110, .T. ) ;
#89310=ORIENTED_EDGE ( 'NONE', *, *, #35060, .T. ) ;
#89311=CIRCLE ( 'NONE', #16125, 0.09999999999999999167 ) ;
#89312=AXIS2_PLACEMENT_3D ( 'NONE', #60802, #58240, #28776 ) ;
#89313=DIRECTION ( 'NONE',  ( 0.000000000000000000, 0.000000000000000000, 1.000000000000000000 ) ) ;
#89314=ORIENTED_EDGE ( 'NONE', *, *, #82134, .T. ) ;
#89315=VERTEX_POINT ( 'NONE', #44865 ) ;
#89316=PLANE ( 'NONE',  #122035 ) ;
#89317=EDGE_CURVE ( 'NONE', #22678, #97846, #63544, .T. ) ;
#89318=EDGE_CURVE ( 'NONE', #2346, #46559, #52101, .T. ) ;
#89320=DIRECTION ( 'NONE',  ( 0.000000000000000000, 0.000000000000000000, 1.000000000000000000 ) ) ;
#89321=DIRECTION ( 'NONE',  ( -0.000000000000000000, -1.000000000000000000, -0.000000000000000000 ) ) ;
#89322=ADVANCED_FACE ( 'NONE', ( #64485 ), #57276, .T. ) ;
#89323=AXIS2_PLACEMENT_3D ( 'NONE', #112320, #110375, #60018 ) ;
#89324=AXIS2_PLACEMENT_3D ( 'NONE', #53611, #103998, #14927 ) ;
#89325=EDGE_LOOP ( 'NONE', ( #116846, #15999 ) ) ;
#89326=EDGE_CURVE ( 'NONE', #99388, #40733, #11301, .T. ) ;
#89327=AXIS2_PLACEMENT_3D ( 'NONE', #89200, #118010, #28359 ) ;
#89328=CARTESIAN_POINT ( 'NONE',  ( -4.400000000000025224, 2.500000000000000000, -0.2464101615137783419 ) ) ;
#89329=ADVANCED_FACE ( 'NONE', ( #93312 ), #17551, .T. ) ;
#89330=FACE_OUTER_BOUND ( 'NONE', #31088, .T. ) ;
#89331=VERTEX_POINT ( 'NONE', #112950 ) ;
#89332=DIRECTION ( 'NONE',  ( -0.000000000000000000, -1.000000000000000000, -0.000000000000000000 ) ) ;
#89333=DIRECTION ( 'NONE',  ( -0.000000000000000000, 1.000000000000000000, -0.000000000000000000 ) ) ;
#89334=EDGE_CURVE ( 'NONE', #96595, #45172, #94936, .T. ) ;
#89335=ORIENTED_EDGE ( 'NONE', *, *, #111164, .F. ) ;
#89336=CONICAL_SURFACE ( 'NONE', #43670, 0.09999999999999999167, 0.003490658503988666988 ) ;
#89337=VERTEX_POINT ( 'NONE', #82202 ) ;
#89338=EDGE_LOOP ( 'NONE', ( #82658, #29060, #59650, #96321 ) ) ;
#89339=DIRECTION ( 'NONE',  ( -0.000000000000000000, 1.000000000000000000, -0.000000000000000000 ) ) ;
#89340=DIRECTION ( 'NONE',  ( -0.000000000000000000, 1.000000000000000000, -0.000000000000000000 ) ) ;
#89341=DIRECTION ( 'NONE',  ( -4.274815082592931898E-19, -0.9999939076577903929, -0.003490651415223739937 ) ) ;
#89342=FACE_BOUND ( 'NONE', #89749, .T. ) ;
#89343=ORIENTED_EDGE ( 'NONE', *, *, #105207, .F. ) ;
#89345=DIRECTION ( 'NONE',  ( 0.000000000000000000, 0.000000000000000000, -1.000000000000000000 ) ) ;
#89346=CARTESIAN_POINT ( 'NONE',  ( -10.00000000000000711, 2.500000000000000000, -3.737306695894645259 ) ) ;
#89347=AXIS2_PLACEMENT_3D ( 'NONE', #62201, #100796, #11129 ) ;
#89348=ORIENTED_EDGE ( 'NONE', *, *, #28275, .F. ) ;
#89349=DIRECTION ( 'NONE',  ( 0.000000000000000000, 1.000000000000000000, 0.000000000000000000 ) ) ;
#89350=CARTESIAN_POINT ( 'NONE',  ( -15.39999999999998082, 12.50000000000000000, 0.6277270498435143509 ) ) ;
#89352=DIRECTION ( 'NONE',  ( 0.000000000000000000, -0.9999939076577903929, 0.003490651415223739937 ) ) ;
#89353=DIRECTION ( 'NONE',  ( -0.000000000000000000, 1.000000000000000000, -0.000000000000000000 ) ) ;
#89354=CARTESIAN_POINT ( 'NONE',  ( -10.85000000000000142, 12.50000000000000000, -5.737276932171709198 ) ) ;
#89355=CARTESIAN_POINT ( 'NONE',  ( 14.79999999999989413, 2.500000000000000000, -0.4464101615137782142 ) ) ;
#89356=CIRCLE ( 'NONE', #120659, 0.06509327318403745899 ) ;
#89357=CARTESIAN_POINT ( 'NONE',  ( 7.499999999999961808, 12.50000000000000000, 4.330127018922196314 ) ) ;
#89358=AXIS2_PLACEMENT_3D ( 'NONE', #65856, #108991, #39656 ) ;
#89359=CONICAL_SURFACE ( 'NONE', #101879, 0.09999999999999982514, 0.003490658503988666988 ) ;
#89360=CIRCLE ( 'NONE', #108132, 0.06509327318403745899 ) ;
#89361=EDGE_LOOP ( 'NONE', ( #84357, #114613 ) ) ;
#89362=ORIENTED_EDGE ( 'NONE', *, *, #28109, .F. ) ;
#89363=ORIENTED_EDGE ( 'NONE', *, *, #111451, .F. ) ;
#89364=ORIENTED_EDGE ( 'NONE', *, *, #92037, .F. ) ;
#89366=CARTESIAN_POINT ( 'NONE',  ( -0.8500000000000382805, 12.50000000000000000, -1.407149913249512663 ) ) ;
#89367=CARTESIAN_POINT ( 'NONE',  ( -4.293440603042597559E-14, 12.50000000000000000, 5.022947341949748790 ) ) ;
#89368=CONICAL_SURFACE ( 'NONE', #87199, 0.09999999999999982514, 0.003490658503988666988 ) ;
#89369=ORIENTED_EDGE ( 'NONE', *, *, #79630, .F. ) ;
#89370=FACE_BOUND ( 'NONE', #11902, .T. ) ;
#89371=DIRECTION ( 'NONE',  ( -0.000000000000000000, 1.000000000000000000, -0.000000000000000000 ) ) ;
#89372=ADVANCED_FACE ( 'NONE', ( #65114 ), #34311, .T. ) ;
#89374=AXIS2_PLACEMENT_3D ( 'NONE', #3727, #51560, #13542 ) ;
#89376=ADVANCED_FACE ( 'NONE', ( #2324 ), #43586, .T. ) ;
#89377=CARTESIAN_POINT ( 'NONE',  ( 3.099999999999943245, 2.500000000000000000, 3.983716857408420076 ) ) ;
#89378=CARTESIAN_POINT ( 'NONE',  ( -8.150000000000012790, 2.500000000000000000, -2.611473670974877592 ) ) ;
#89379=DIRECTION ( 'NONE',  ( 0.000000000000000000, 0.000000000000000000, 1.000000000000000000 ) ) ;
#89380=CARTESIAN_POINT ( 'NONE',  ( -10.65000000000000391, 12.50000000000000000, -1.818653347947322141 ) ) ;
#89381=ORIENTED_EDGE ( 'NONE', *, *, #100842, .T. ) ;
#89382=EDGE_CURVE ( 'NONE', #24998, #45239, #89673, .T. ) ;
#89383=ORIENTED_EDGE ( 'NONE', *, *, #4191, .T. ) ;
#89384=ORIENTED_EDGE ( 'NONE', *, *, #40358, .F. ) ;
#89385=ORIENTED_EDGE ( 'NONE', *, *, #43511, .F. ) ;
#89386=CARTESIAN_POINT ( 'NONE',  ( 12.31005523242794375, 2.499999999999999112, 7.488833079370742496 ) ) ;
#89387=CARTESIAN_POINT ( 'NONE',  ( 11.69999999999990870, 12.50000000000000000, 4.330127018922196314 ) ) ;
#89388=ORIENTED_EDGE ( 'NONE', *, *, #124788, .T. ) ;
#89389=CONICAL_SURFACE ( 'NONE', #93498, 0.1000000000000002554, 0.003490658503988666988 ) ;
#89390=CARTESIAN_POINT ( 'NONE',  ( -2.300000000000032685, 12.50000000000000000, -0.3464101615137783474 ) ) ;
#89391=DIRECTION ( 'NONE',  ( -4.274815082592931898E-19, -0.9999939076577903929, -0.003490651415223739937 ) ) ;
#89392=DIRECTION ( 'NONE',  ( -0.000000000000000000, -1.000000000000000000, -0.000000000000000000 ) ) ;
#89394=CARTESIAN_POINT ( 'NONE',  ( -2.900000000000029665, 2.500000000000000000, 3.537306695894645081 ) ) ;
#89395=DIRECTION ( 'NONE',  ( 0.000000000000000000, 0.000000000000000000, 1.000000000000000000 ) ) ;
#89396=DIRECTION ( 'NONE',  ( 0.000000000000000000, 1.000000000000000000, 0.000000000000000000 ) ) ;
#89397=ORIENTED_EDGE ( 'NONE', *, *, #114497, .T. ) ;
#89398=CARTESIAN_POINT ( 'NONE',  ( 5.599999999999933031, 2.500000000000000000, -0.3464101615137783474 ) ) ;
#89399=VERTEX_POINT ( 'NONE', #17961 ) ;
#89400=AXIS2_PLACEMENT_3D ( 'NONE', #52594, #32346, #72889 ) ;
#89401=EDGE_LOOP ( 'NONE', ( #20971, #49376, #84206, #43635 ) ) ;
#89402=DIRECTION ( 'NONE',  ( 0.000000000000000000, -0.9999939076577903929, 0.003490651415223739937 ) ) ;
#89403=DIRECTION ( 'NONE',  ( 0.000000000000000000, 0.000000000000000000, -1.000000000000000000 ) ) ;
#89404=DIRECTION ( 'NONE',  ( 0.000000000000000000, 0.000000000000000000, 1.000000000000000000 ) ) ;
#89405=ORIENTED_EDGE ( 'NONE', *, *, #32016, .F. ) ;
#89406=ORIENTED_EDGE ( 'NONE', *, *, #104529, .F. ) ;
#89407=ADVANCED_FACE ( 'NONE', ( #27776 ), #12296, .T. ) ;
#89408=DIRECTION ( 'NONE',  ( -0.000000000000000000, -1.000000000000000000, -0.000000000000000000 ) ) ;
#89409=CIRCLE ( 'NONE', #66321, 0.06509327318403745899 ) ;
#89410=AXIS2_PLACEMENT_3D ( 'NONE', #61718, #112097, #32269 ) ;
#89411=CARTESIAN_POINT ( 'NONE',  ( 6.449999999999928235, 2.500000000000000000, 2.511473670974873507 ) ) ;
#89412=DIRECTION ( 'NONE',  ( -0.000000000000000000, 1.000000000000000000, -0.000000000000000000 ) ) ;
#89413=CARTESIAN_POINT ( 'NONE',  ( 4.149999999999939959, 12.50000000000000000, -6.495190528383302464 ) ) ;
#89414=ORIENTED_EDGE ( 'NONE', *, *, #79572, .F. ) ;
#89415=FACE_OUTER_BOUND ( 'NONE', #36502, .T. ) ;
#89416=EDGE_LOOP ( 'NONE', ( #32549, #52925, #14419, #66026 ) ) ;
#89417=DIRECTION ( 'NONE',  ( 0.000000000000000000, 1.000000000000000000, 0.000000000000000000 ) ) ;
#89418=CONICAL_SURFACE ( 'NONE', #43464, 0.1000000000000000472, 0.003490658503988666988 ) ;
#89419=ORIENTED_EDGE ( 'NONE', *, *, #6107, .T. ) ;
#89420=CARTESIAN_POINT ( 'NONE',  ( 43.29488993686067033, -3.510952053399744255, 3.940495137596863984 ) ) ;
#89421=FACE_OUTER_BOUND ( 'NONE', #97490, .T. ) ;
#89422=ADVANCED_FACE ( 'NONE', ( #45514 ), #78189, .T. ) ;
#89423=AXIS2_PLACEMENT_3D ( 'NONE', #4250, #35675, #35047 ) ;
#89424=EDGE_CURVE ( 'NONE', #1125, #70010, #116800, .T. ) ;
#89425=DIRECTION ( 'NONE',  ( 0.000000000000000000, 1.000000000000000000, 0.000000000000000000 ) ) ;
#89426=EDGE_LOOP ( 'NONE', ( #38034, #68941 ) ) ;
#89427=DIRECTION ( 'NONE',  ( -0.000000000000000000, -1.000000000000000000, -0.000000000000000000 ) ) ;
#89428=CIRCLE ( 'NONE', #51781, 0.1000000000000002554 ) ;
#89429=VERTEX_POINT ( 'NONE', #85418 ) ;
#89430=ORIENTED_EDGE ( 'NONE', *, *, #24125, .F. ) ;
#89431=EDGE_CURVE ( 'NONE', #76810, #13985, #33260, .T. ) ;
#89432=CARTESIAN_POINT ( 'NONE',  ( -13.74999999999998757, 2.500000000000000000, -2.857883832488651521 ) ) ;
#89433=CARTESIAN_POINT ( 'NONE',  ( 3.349999999999943689, 12.50000000000000000, 2.165063509461097713 ) ) ;
#89434=CARTESIAN_POINT ( 'NONE',  ( 19.01901804971413767, 2.576149587736929369, 2.431039412660860766 ) ) ;
#89435=FACE_OUTER_BOUND ( 'NONE', #57711, .T. ) ;
#89436=CONICAL_SURFACE ( 'NONE', #81035, 0.1000000000000000472, 0.003490658503988666988 ) ;
#89437=CARTESIAN_POINT ( 'NONE',  ( 3.949999999999941558, 2.500000000000000000, -6.148780366869526226 ) ) ;
#89438=AXIS2_PLACEMENT_3D ( 'NONE', #91655, #81204, #123057 ) ;
#89439=DIRECTION ( 'NONE',  ( 0.000000000000000000, 0.000000000000000000, 1.000000000000000000 ) ) ;
#89440=VECTOR ( 'NONE', #66289, 1000.000000000000000 ) ;
#89441=CARTESIAN_POINT ( 'NONE',  ( -8.100000000000013856, 12.50000000000000000, -3.983716857408426293 ) ) ;
#89442=LINE ( 'NONE', #129398, #63837 ) ;
#89443=CARTESIAN_POINT ( 'NONE',  ( -2.500000000000030642, 2.500000000000000000, -0.6928203230275541413 ) ) ;
#89444=CIRCLE ( 'NONE', #112442, 0.09999999999999999167 ) ;
#89445=AXIS2_PLACEMENT_3D ( 'NONE', #91954, #21940, #93249 ) ;
#89446=VECTOR ( 'NONE', #87537, 1000.000000000000000 ) ;
#89447=ORIENTED_EDGE ( 'NONE', *, *, #73825, .F. ) ;
#89448=CARTESIAN_POINT ( 'NONE',  ( -13.34999999999999076, 2.500000000000000000, 2.757883832488653209 ) ) ;
#89449=AXIS2_PLACEMENT_3D ( 'NONE', #97292, #38395, #19359 ) ;
#89450=CARTESIAN_POINT ( 'NONE',  ( -11.44999999999999751, 2.500000000000000000, 2.411473670974873862 ) ) ;
#89451=DIRECTION ( 'NONE',  ( -0.000000000000000000, 1.000000000000000000, -0.000000000000000000 ) ) ;
#89452=CARTESIAN_POINT ( 'NONE',  ( 3.349999999999943689, 2.500000000000000000, 2.265063509461097357 ) ) ;
#89453=PLANE ( 'NONE',  #108680 ) ;
#89454=ORIENTED_EDGE ( 'NONE', *, *, #88631, .T. ) ;
#89455=DIRECTION ( 'NONE',  ( -0.000000000000000000, 1.000000000000000000, -0.000000000000000000 ) ) ;
#89456=ADVANCED_FACE ( 'NONE', ( #86038 ), #27146, .T. ) ;
#89457=CIRCLE ( 'NONE', #87299, 0.09999999999999982514 ) ;
#89458=AXIS2_PLACEMENT_3D ( 'NONE', #18702, #58647, #128700 ) ;
#89459=DIRECTION ( 'NONE',  ( 0.000000000000000000, 1.000000000000000000, 0.000000000000000000 ) ) ;
#89460=FACE_OUTER_BOUND ( 'NONE', #20832, .T. ) ;
#89461=VERTEX_POINT ( 'NONE', #75584 ) ;
#89463=EDGE_CURVE ( 'NONE', #129515, #95931, #118912, .T. ) ;
#89464=ORIENTED_EDGE ( 'NONE', *, *, #99337, .T. ) ;
#89465=PLANE ( 'NONE',  #19678 ) ;
#89466=ORIENTED_EDGE ( 'NONE', *, *, #103004, .F. ) ;
#89467=EDGE_LOOP ( 'NONE', ( #75715, #105419 ) ) ;
#89468=ORIENTED_EDGE ( 'NONE', *, *, #125179, .F. ) ;
#89469=CARTESIAN_POINT ( 'NONE',  ( 9.349999999999919709, 2.500000000000000000, -6.741600689897078169 ) ) ;
#89470=EDGE_CURVE ( 'NONE', #124980, #76747, #97811, .T. ) ;
#89471=EDGE_CURVE ( 'NONE', #46350, #93541, #98067, .T. ) ;
#89472=EDGE_CURVE ( 'NONE', #5769, #114671, #45764, .T. ) ;
#89474=DIRECTION ( 'NONE',  ( 0.000000000000000000, 0.000000000000000000, 1.000000000000000000 ) ) ;
#89475=DIRECTION ( 'NONE',  ( 0.000000000000000000, 1.000000000000000000, 0.000000000000000000 ) ) ;
#89476=ORIENTED_EDGE ( 'NONE', *, *, #67845, .T. ) ;
#89477=ADVANCED_FACE ( 'NONE', ( #5556 ), #31197, .T. ) ;
#89478=CARTESIAN_POINT ( 'NONE',  ( -5.600000000000020073, 12.50000000000000000, 3.983716857408420964 ) ) ;
#89479=ORIENTED_EDGE ( 'NONE', *, *, #13180, .F. ) ;
#89480=DIRECTION ( 'NONE',  ( 0.000000000000000000, 1.000000000000000000, 0.000000000000000000 ) ) ;
#89481=AXIS2_PLACEMENT_3D ( 'NONE', #17555, #88209, #57502 ) ;
#89482=CARTESIAN_POINT ( 'NONE',  ( 19.72570408286463106, 0.6078483229320776893, 4.299616118078733784 ) ) ;
#89483=CARTESIAN_POINT ( 'NONE',  ( -0.8500000000000382805, 2.500000000000000000, -5.702370205355749455 ) ) ;
#89484=DIRECTION ( 'NONE',  ( 0.000000000000000000, 0.000000000000000000, 1.000000000000000000 ) ) ;
#89485=EDGE_CURVE ( 'NONE', #126098, #123229, #83424, .T. ) ;
#89486=ORIENTED_EDGE ( 'NONE', *, *, #45344, .F. ) ;
#89487=CONICAL_SURFACE ( 'NONE', #12114, 0.09999999999999982514, 0.003490658503988666988 ) ;
#89488=CIRCLE ( 'NONE', #33081, 0.06509327318403745899 ) ;
#89489=ORIENTED_EDGE ( 'NONE', *, *, #59632, .F. ) ;
#89490=EDGE_LOOP ( 'NONE', ( #34297, #10494, #43088, #35789 ) ) ;
#89491=VERTEX_POINT ( 'NONE', #46794 ) ;
#89492=ORIENTED_EDGE ( 'NONE', *, *, #26434, .F. ) ;
#89493=DIRECTION ( 'NONE',  ( 0.000000000000000000, 0.000000000000000000, -1.000000000000000000 ) ) ;
#89494=CARTESIAN_POINT ( 'NONE',  ( -1.700000000000035261, 2.500000000000000000, 4.330127018922196314 ) ) ;
#89495=CARTESIAN_POINT ( 'NONE',  ( -12.49999999999999289, 2.500000000000000000, 5.022947341949748790 ) ) ;
#89496=FACE_BOUND ( 'NONE', #86346, .T. ) ;
#89497=CARTESIAN_POINT ( 'NONE',  ( 3.749999999999944045, 2.500000000000000000, -2.857883832488653741 ) ) ;
#89498=CARTESIAN_POINT ( 'NONE',  ( -8.350000000000013856, 2.500000000000000000, -7.088010851410848190 ) ) ;
#89499=CIRCLE ( 'NONE', #47742, 0.09999999999999999167 ) ;
#89500=DIRECTION ( 'NONE',  ( 0.000000000000000000, 1.000000000000000000, 0.000000000000000000 ) ) ;
#89501=FACE_OUTER_BOUND ( 'NONE', #121094, .T. ) ;
#89502=CARTESIAN_POINT ( 'NONE',  ( 10.64999999999990976, 2.500000000000000000, -6.741600689897077281 ) ) ;
#89503=CARTESIAN_POINT ( 'NONE',  ( -10.20000000000000462, 2.500000000000000000, 0.3464101615137735735 ) ) ;
#89504=CARTESIAN_POINT ( 'NONE',  ( -3.350000000000028511, 2.500000000000000000, 1.472243186433545459 ) ) ;
#89505=AXIS2_PLACEMENT_3D ( 'NONE', #113184, #34663, #86297 ) ;
#89506=LINE ( 'NONE', #99338, #70265 ) ;
#89507=ORIENTED_EDGE ( 'NONE', *, *, #71456, .F. ) ;
#89508=ORIENTED_EDGE ( 'NONE', *, *, #105848, .T. ) ;
#89509=ORIENTED_EDGE ( 'NONE', *, *, #28852, .F. ) ;
#89510=ORIENTED_EDGE ( 'NONE', *, *, #53399, .T. ) ;
#89511=CIRCLE ( 'NONE', #97914, 0.06509327318403745899 ) ;
#89512=DIRECTION ( 'NONE',  ( 0.000000000000000000, 0.000000000000000000, 1.000000000000000000 ) ) ;
#89513=CARTESIAN_POINT ( 'NONE',  ( 7.949999999999925571, 12.50000000000000000, -6.495190528383302464 ) ) ;
#89514=FACE_BOUND ( 'NONE', #115004, .T. ) ;
#89515=DIRECTION ( 'NONE',  ( -0.000000000000000000, 1.000000000000000000, -0.000000000000000000 ) ) ;
#89516=AXIS2_PLACEMENT_3D ( 'NONE', #41168, #79777, #50318 ) ;
#89517=EDGE_CURVE ( 'NONE', #17700, #23794, #79220, .T. ) ;
#89518=EDGE_LOOP ( 'NONE', ( #101188, #29358 ) ) ;
#89519=CARTESIAN_POINT ( 'NONE',  ( 9.149999999999920419, 2.500000000000000000, -5.702370205355749455 ) ) ;
#89520=DIRECTION ( 'NONE',  ( -4.274815082592931898E-19, -0.9999939076577903929, -0.003490651415223739937 ) ) ;
#89521=DIRECTION ( 'NONE',  ( 0.000000000000000000, 0.000000000000000000, -1.000000000000000000 ) ) ;
#89522=CARTESIAN_POINT ( 'NONE',  ( -9.350000000000006750, 12.50000000000000000, -1.753560074763288457 ) ) ;
#89523=AXIS2_PLACEMENT_3D ( 'NONE', #75535, #97770, #8091 ) ;
#89524=EDGE_LOOP ( 'NONE', ( #25018, #36566 ) ) ;
#89525=AXIS2_PLACEMENT_3D ( 'NONE', #72361, #35026, #3606 ) ;
#89526=DIRECTION ( 'NONE',  ( 0.000000000000000000, -0.000000000000000000, 1.000000000000000000 ) ) ;
#89527=ADVANCED_FACE ( 'NONE', ( #38265 ), #93879, .T. ) ;
#89528=AXIS2_PLACEMENT_3D ( 'NONE', #111342, #30897, #100265 ) ;
#89529=ORIENTED_EDGE ( 'NONE', *, *, #3179, .F. ) ;
#89530=VERTEX_POINT ( 'NONE', #95248 ) ;
#89531=CARTESIAN_POINT ( 'NONE',  ( 5.649999999999936406, 12.50000000000000000, -6.906693963081115051 ) ) ;
#89532=DIRECTION ( 'NONE',  ( 0.000000000000000000, 0.000000000000000000, 1.000000000000000000 ) ) ;
#89533=VERTEX_POINT ( 'NONE', #65767 ) ;
#89534=DIRECTION ( 'NONE',  ( 0.000000000000000000, 0.000000000000000000, 1.000000000000000000 ) ) ;
#89536=ORIENTED_EDGE ( 'NONE', *, *, #125660, .F. ) ;
#89537=CARTESIAN_POINT ( 'NONE',  ( -11.69999999999999929, 12.50000000000000000, -4.330127018922198978 ) ) ;
#89538=ORIENTED_EDGE ( 'NONE', *, *, #71889, .F. ) ;
#89539=AXIS2_PLACEMENT_3D ( 'NONE', #123162, #111382, #61676 ) ;
#89540=FACE_OUTER_BOUND ( 'NONE', #103697, .T. ) ;
#89541=ORIENTED_EDGE ( 'NONE', *, *, #62258, .T. ) ;
#89542=DIRECTION ( 'NONE',  ( 0.000000000000000000, 1.000000000000000000, 0.000000000000000000 ) ) ;
#89543=FACE_BOUND ( 'NONE', #78427, .T. ) ;
#89544=AXIS2_PLACEMENT_3D ( 'NONE', #26324, #21486, #7298 ) ;
#89545=VECTOR ( 'NONE', #124253, 1000.000000000000000 ) ;
#89546=ORIENTED_EDGE ( 'NONE', *, *, #119017, .F. ) ;
#89548=ORIENTED_EDGE ( 'NONE', *, *, #96140, .F. ) ;
#89549=DIRECTION ( 'NONE',  ( 0.000000000000000000, 0.000000000000000000, 1.000000000000000000 ) ) ;
#89550=CARTESIAN_POINT ( 'NONE',  ( -1.650000000000034328, 12.50000000000000000, -6.430097255199264339 ) ) ;
#89553=CARTESIAN_POINT ( 'NONE',  ( 7.099999999999925926, 2.500000000000000000, 0.5928203230275495006 ) ) ;
#89554=DIRECTION ( 'NONE',  ( 0.000000000000000000, 0.000000000000000000, -1.000000000000000000 ) ) ;
#89555=ORIENTED_EDGE ( 'NONE', *, *, #8606, .T. ) ;
#89556=ORIENTED_EDGE ( 'NONE', *, *, #60791, .T. ) ;
#89557=ADVANCED_FACE ( 'NONE', ( #16655 ), #8179, .T. ) ;
#89558=ORIENTED_EDGE ( 'NONE', *, *, #14084, .F. ) ;
#89559=CARTESIAN_POINT ( 'NONE',  ( 0.8499999999999545697, 2.500000000000000000, 2.857883832488649301 ) ) ;
#89560=CARTESIAN_POINT ( 'NONE',  ( -2.700000000000031264, 12.50000000000000000, 4.741630453620009789 ) ) ;
#89561=CARTESIAN_POINT ( 'NONE',  ( -7.100000000000017408, 2.500000000000000000, -5.022947341949754119 ) ) ;
#89562=CIRCLE ( 'NONE', #102086, 0.09999999999999999167 ) ;
#89563=VERTEX_POINT ( 'NONE', #96502 ) ;
#89564=ORIENTED_EDGE ( 'NONE', *, *, #119416, .T. ) ;
#89565=EDGE_LOOP ( 'NONE', ( #102615, #101690 ) ) ;
#89566=DIRECTION ( 'NONE',  ( 0.000000000000000000, -0.9999939076577903929, 0.003490651415223739937 ) ) ;
#89567=ORIENTED_EDGE ( 'NONE', *, *, #67389, .F. ) ;
#89568=DIRECTION ( 'NONE',  ( 0.000000000000000000, 0.000000000000000000, 1.000000000000000000 ) ) ;
#89569=EDGE_CURVE ( 'NONE', #91861, #87824, #37454, .T. ) ;
#89570=CONICAL_SURFACE ( 'NONE', #33147, 0.1000000000000002554, 0.003490658503988666988 ) ;
#89571=VECTOR ( 'NONE', #6182, 1000.000000000000000 ) ;
#89572=CARTESIAN_POINT ( 'NONE',  ( -11.24999999999996270, 12.50000000000000000, 2.165063509461097713 ) ) ;
#89574=AXIS2_PLACEMENT_3D ( 'NONE', #97451, #7773, #68634 ) ;
#89575=PLANE ( 'NONE',  #109186 ) ;
#89576=LINE ( 'NONE', #79754, #19987 ) ;
#89577=CARTESIAN_POINT ( 'NONE',  ( -12.09999999999999609, 2.500000000000000000, -5.122947341949751987 ) ) ;
#89578=EDGE_CURVE ( 'NONE', #13125, #119700, #49383, .T. ) ;
#89579=EDGE_CURVE ( 'NONE', #96780, #3042, #47918, .T. ) ;
#89580=CARTESIAN_POINT ( 'NONE',  ( -8.550000000000011369, 12.50000000000000000, -2.446380397790840266 ) ) ;
#89581=VECTOR ( 'NONE', #65563, 1000.000000000000000 ) ;
#89582=ORIENTED_EDGE ( 'NONE', *, *, #22732, .F. ) ;
#89583=CONICAL_SURFACE ( 'NONE', #12197, 0.09999999999999982514, 0.003490658503988666988 ) ;
#89584=ORIENTED_EDGE ( 'NONE', *, *, #17803, .F. ) ;
#89585=VECTOR ( 'NONE', #45211, 1000.000000000000000 ) ;
#89586=CARTESIAN_POINT ( 'NONE',  ( 9.149999999999916866, 2.500000000000000000, 5.802370205355744659 ) ) ;
#89588=LINE ( 'NONE', #122115, #25666 ) ;
#89589=ORIENTED_EDGE ( 'NONE', *, *, #109184, .F. ) ;
#89590=ORIENTED_EDGE ( 'NONE', *, *, #31645, .F. ) ;
#89591=ADVANCED_FACE ( 'NONE', ( #78845 ), #24919, .T. ) ;
#89593=DIRECTION ( 'NONE',  ( -0.000000000000000000, 1.000000000000000000, -0.000000000000000000 ) ) ;
#89594=DIRECTION ( 'NONE',  ( -4.274815082592931898E-19, -0.9999939076577903929, -0.003490651415223739937 ) ) ;
#89595=AXIS2_PLACEMENT_3D ( 'NONE', #103178, #3684, #16058 ) ;
#89596=CARTESIAN_POINT ( 'NONE',  ( -4.800000000000024691, 12.50000000000000000, 0.4115034346978109769 ) ) ;
#89597=AXIS2_PLACEMENT_3D ( 'NONE', #51776, #32152, #91698 ) ;
#89598=DIRECTION ( 'NONE',  ( 0.000000000000000000, 1.000000000000000000, 0.000000000000000000 ) ) ;
#89599=PLANE ( 'NONE',  #88683 ) ;
#89600=FACE_OUTER_BOUND ( 'NONE', #124540, .T. ) ;
#89601=DIRECTION ( 'NONE',  ( 0.000000000000000000, 0.000000000000000000, 1.000000000000000000 ) ) ;
#89602=AXIS2_PLACEMENT_3D ( 'NONE', #66659, #106592, #56825 ) ;
#89603=VERTEX_POINT ( 'NONE', #120041 ) ;
#89604=ORIENTED_EDGE ( 'NONE', *, *, #65176, .T. ) ;
#89606=AXIS2_PLACEMENT_3D ( 'NONE', #59696, #62256, #40697 ) ;
#89607=ORIENTED_EDGE ( 'NONE', *, *, #41588, .F. ) ;
#89608=VERTEX_POINT ( 'NONE', #18610 ) ;
#89609=DIRECTION ( 'NONE',  ( -0.000000000000000000, 1.000000000000000000, -0.000000000000000000 ) ) ;
#89610=CARTESIAN_POINT ( 'NONE',  ( -10.40000000000000213, 2.500000000000000000, -0.7928203230275542301 ) ) ;
#89611=VECTOR ( 'NONE', #55478, 1000.000000000000000 ) ;
#89612=ORIENTED_EDGE ( 'NONE', *, *, #49604, .F. ) ;
#89614=ADVANCED_FACE ( 'NONE', ( #61111 ), #118741, .T. ) ;
#89615=FACE_OUTER_BOUND ( 'NONE', #100189, .T. ) ;
#89616=CARTESIAN_POINT ( 'NONE',  ( 0.5999999999999560130, 2.500000000000000000, -3.883716857408426648 ) ) ;
#89617=CARTESIAN_POINT ( 'NONE',  ( 11.44999999999990514, 12.50000000000000000, 2.511473670974873507 ) ) ;
#89618=ORIENTED_EDGE ( 'NONE', *, *, #75141, .F. ) ;
#89619=DIRECTION ( 'NONE',  ( -0.000000000000000000, 1.000000000000000000, -0.000000000000000000 ) ) ;
#89620=EDGE_CURVE ( 'NONE', #89736, #116685, #50648, .T. ) ;
#89621=CARTESIAN_POINT ( 'NONE',  ( -13.09999999999999254, 12.50000000000000000, -0.2813168883297366696 ) ) ;
#89622=EDGE_LOOP ( 'NONE', ( #93196, #39897, #109388, #91744 ) ) ;
#89623=AXIS2_PLACEMENT_3D ( 'NONE', #3348, #43288, #49093 ) ;
#89624=ORIENTED_EDGE ( 'NONE', *, *, #121521, .T. ) ;
#89626=VERTEX_POINT ( 'NONE', #30388 ) ;
#89627=DIRECTION ( 'NONE',  ( 0.000000000000000000, 1.000000000000000000, 0.000000000000000000 ) ) ;
#89628=EDGE_CURVE ( 'NONE', #39021, #114247, #127333, .T. ) ;
#89629=CIRCLE ( 'NONE', #66540, 0.1000000000000002554 ) ;
#89630=ADVANCED_FACE ( 'NONE', ( #110220 ), #88640, .T. ) ;
#89631=EDGE_CURVE ( 'NONE', #126381, #20628, #16488, .T. ) ;
#89632=CARTESIAN_POINT ( 'NONE',  ( -13.54999999999998828, 2.500000000000000000, -2.411473670974875638 ) ) ;
#89633=DIRECTION ( 'NONE',  ( 0.000000000000000000, 0.000000000000000000, 1.000000000000000000 ) ) ;
#89634=AXIS2_PLACEMENT_3D ( 'NONE', #21685, #96048, #83809 ) ;
#89635=VECTOR ( 'NONE', #30109, 1000.000000000000000 ) ;
#89636=EDGE_CURVE ( 'NONE', #8732, #43124, #41668, .T. ) ;
#89637=VERTEX_POINT ( 'NONE', #129242 ) ;
#89638=DIRECTION ( 'NONE',  ( 0.000000000000000000, 1.000000000000000000, 0.000000000000000000 ) ) ;
#89639=DIRECTION ( 'NONE',  ( 0.000000000000000000, 0.000000000000000000, -1.000000000000000000 ) ) ;
#89640=VECTOR ( 'NONE', #112388, 1000.000000000000000 ) ;
#89641=FACE_OUTER_BOUND ( 'NONE', #3626, .T. ) ;
#89642=DIRECTION ( 'NONE',  ( 0.000000000000000000, 0.000000000000000000, 1.000000000000000000 ) ) ;
#89644=VERTEX_POINT ( 'NONE', #19912 ) ;
#89645=CIRCLE ( 'NONE', #106362, 0.06509327318403741736 ) ;
#89646=AXIS2_PLACEMENT_3D ( 'NONE', #12976, #92868, #83048 ) ;
#89647=ADVANCED_FACE ( 'NONE', ( #91222 ), #108440, .T. ) ;
#89649=EDGE_LOOP ( 'NONE', ( #954, #83570, #68231, #103432 ) ) ;
#89650=VERTEX_POINT ( 'NONE', #902 ) ;
#89651=DIRECTION ( 'NONE',  ( 0.000000000000000000, 1.000000000000000000, 0.000000000000000000 ) ) ;
#89652=CARTESIAN_POINT ( 'NONE',  ( 8.749999999999923617, 12.50000000000000000, 1.472243186433545459 ) ) ;
#89653=FACE_BOUND ( 'NONE', #22176, .T. ) ;
#89654=CARTESIAN_POINT ( 'NONE',  ( -3.350000000000028511, 12.50000000000000000, -2.857883832488653741 ) ) ;
#89655=LINE ( 'NONE', #18320, #59126 ) ;
#89656=CARTESIAN_POINT ( 'NONE',  ( -9.150000000000009237, 12.50000000000000000, -2.165063509461101710 ) ) ;
#89657=CIRCLE ( 'NONE', #43712, 0.09999999999999982514 ) ;
#89658=ORIENTED_EDGE ( 'NONE', *, *, #99843, .F. ) ;
#89659=DIRECTION ( 'NONE',  ( 0.000000000000000000, 0.000000000000000000, -1.000000000000000000 ) ) ;
#89660=CARTESIAN_POINT ( 'NONE',  ( 8.149999999999923972, 12.50000000000000000, 2.446380397790835826 ) ) ;
#89661=PLANE ( 'NONE',  #80033 ) ;
#89662=FACE_OUTER_BOUND ( 'NONE', #26539, .T. ) ;
#89663=ORIENTED_EDGE ( 'NONE', *, *, #14070, .T. ) ;
#89664=CARTESIAN_POINT ( 'NONE',  ( -11.25000000000000000, 12.50000000000000000, -7.188010851410850499 ) ) ;
#89665=CIRCLE ( 'NONE', #81259, 0.1000000000000002554 ) ;
#89666=CARTESIAN_POINT ( 'NONE',  ( -12.04999999999999538, 12.50000000000000000, 2.165063509461097713 ) ) ;
#89667=ORIENTED_EDGE ( 'NONE', *, *, #128052, .T. ) ;
#89669=DIRECTION ( 'NONE',  ( 0.000000000000000000, -0.000000000000000000, 1.000000000000000000 ) ) ;
#89670=DIRECTION ( 'NONE',  ( 0.000000000000000000, 0.000000000000000000, -1.000000000000000000 ) ) ;
#89671=FACE_BOUND ( 'NONE', #126239, .T. ) ;
#89672=CARTESIAN_POINT ( 'NONE',  ( -0.6000000000000323963, 2.500000000000000000, 0.2464101615137759549 ) ) ;
#89673=CIRCLE ( 'NONE', #85456, 7.500000000000000000 ) ;
#89674=CIRCLE ( 'NONE', #56208, 0.06509327318403745899 ) ;
#89675=DIRECTION ( 'NONE',  ( 0.000000000000000000, 0.000000000000000000, -1.000000000000000000 ) ) ;
#89676=EDGE_CURVE ( 'NONE', #40679, #11966, #19236, .T. ) ;
#89677=ORIENTED_EDGE ( 'NONE', *, *, #110304, .F. ) ;
#89678=FACE_OUTER_BOUND ( 'NONE', #113917, .T. ) ;
#89680=AXIS2_PLACEMENT_3D ( 'NONE', #91269, #31710, #120726 ) ;
#89681=ORIENTED_EDGE ( 'NONE', *, *, #106889, .F. ) ;
#89683=PLANE ( 'NONE',  #86663 ) ;
#89684=EDGE_CURVE ( 'NONE', #42781, #41615, #114793, .T. ) ;
#89685=DIRECTION ( 'NONE',  ( 0.000000000000000000, 0.000000000000000000, 1.000000000000000000 ) ) ;
#89686=DIRECTION ( 'NONE',  ( -0.000000000000000000, -1.000000000000000000, -0.000000000000000000 ) ) ;
#89687=CIRCLE ( 'NONE', #99884, 0.06509327318403745899 ) ;
#89688=VERTEX_POINT ( 'NONE', #41504 ) ;
#89689=FACE_OUTER_BOUND ( 'NONE', #498, .T. ) ;
#89690=CARTESIAN_POINT ( 'NONE',  ( 8.749999999999957367, 12.50000000000000000, -6.560283801567339701 ) ) ;
#89691=DIRECTION ( 'NONE',  ( 0.000000000000000000, 1.000000000000000000, 0.000000000000000000 ) ) ;
#89692=CIRCLE ( 'NONE', #45882, 0.06509327318403745899 ) ;
#89693=DIRECTION ( 'NONE',  ( -0.000000000000000000, 1.000000000000000000, -0.000000000000000000 ) ) ;
#89694=ORIENTED_EDGE ( 'NONE', *, *, #86245, .T. ) ;
#89695=ORIENTED_EDGE ( 'NONE', *, *, #116820, .F. ) ;
#89696=CARTESIAN_POINT ( 'NONE',  ( 0.8499999999999545697, 12.50000000000000000, -1.407149913249512663 ) ) ;
#89697=EDGE_LOOP ( 'NONE', ( #93274, #120748, #71765, #36286 ) ) ;
#89698=CARTESIAN_POINT ( 'NONE',  ( -6.650000000000014566, 12.50000000000000000, 6.495190528383297135 ) ) ;
#89699=CARTESIAN_POINT ( 'NONE',  ( 17.50000000000000000, -2.500000000000000000, 4.000000000000001776 ) ) ;
#89700=DIRECTION ( 'NONE',  ( 0.000000000000000000, 0.000000000000000000, 1.000000000000000000 ) ) ;
#89701=ORIENTED_EDGE ( 'NONE', *, *, #54398, .F. ) ;
#89702=AXIS2_PLACEMENT_3D ( 'NONE', #55946, #85411, #96498 ) ;
#89703=LINE ( 'NONE', #68120, #60026 ) ;
#89704=CARTESIAN_POINT ( 'NONE',  ( -5.850000000000018296, 2.500000000000000000, 2.857883832488649301 ) ) ;
#89705=CARTESIAN_POINT ( 'NONE',  ( 5.599999999999933031, 2.500000000000000000, 0.3464101615137735735 ) ) ;
#89707=DIRECTION ( 'NONE',  ( 0.000000000000000000, 1.000000000000000000, 0.000000000000000000 ) ) ;
#89708=AXIS2_PLACEMENT_3D ( 'NONE', #49358, #89255, #129214 ) ;
#89709=DIRECTION ( 'NONE',  ( -0.000000000000000000, 1.000000000000000000, -0.000000000000000000 ) ) ;
#89710=CIRCLE ( 'NONE', #106433, 0.09999999999999982514 ) ;
#89711=ORIENTED_EDGE ( 'NONE', *, *, #23443, .T. ) ;
#89712=ORIENTED_EDGE ( 'NONE', *, *, #90322, .F. ) ;
#89713=CARTESIAN_POINT ( 'NONE',  ( 4.999999999999938716, 12.50000000000000000, -4.957854068765716882 ) ) ;
#89714=ORIENTED_EDGE ( 'NONE', *, *, #71633, .T. ) ;
#89715=DIRECTION ( 'NONE',  ( 0.000000000000000000, 0.000000000000000000, 1.000000000000000000 ) ) ;
#89716=ORIENTED_EDGE ( 'NONE', *, *, #128990, .F. ) ;
#89717=ORIENTED_EDGE ( 'NONE', *, *, #63116, .T. ) ;
#89718=ORIENTED_EDGE ( 'NONE', *, *, #64217, .F. ) ;
#89719=FACE_OUTER_BOUND ( 'NONE', #20875, .T. ) ;
#89720=FACE_OUTER_BOUND ( 'NONE', #15808, .T. ) ;
#89721=ADVANCED_FACE ( 'NONE', ( #99115 ), #87598, .T. ) ;
#89722=CARTESIAN_POINT ( 'NONE',  ( 10.39999999999991154, 12.50000000000000000, -3.702399969078687292 ) ) ;
#89724=CIRCLE ( 'NONE', #37508, 0.1000000000000002554 ) ;
#89725=CARTESIAN_POINT ( 'NONE',  ( -10.40000000000000391, 2.500000000000000000, -3.637306695894645614 ) ) ;
#89726=CARTESIAN_POINT ( 'NONE',  ( 8.149999999999920419, 2.500000000000000000, -1.718653347947325827 ) ) ;
#89727=CARTESIAN_POINT ( 'NONE',  ( 11.04999999999991012, 2.500000000000000000, 6.741600689897071952 ) ) ;
#89729=DIRECTION ( 'NONE',  ( 0.000000000000000000, 1.000000000000000000, 0.000000000000000000 ) ) ;
#89730=CONICAL_SURFACE ( 'NONE', #123186, 0.1000000000000002554, 0.003490658503988666988 ) ;
#89731=EDGE_CURVE ( 'NONE', #50580, #60734, #1923, .T. ) ;
#89732=EDGE_CURVE ( 'NONE', #93869, #118548, #102963, .T. ) ;
#89733=CARTESIAN_POINT ( 'NONE',  ( 12.09999999999990550, 2.500000000000000000, 3.637306695894644726 ) ) ;
#89734=VERTEX_POINT ( 'NONE', #32967 ) ;
#89735=CIRCLE ( 'NONE', #98046, 0.06509327318403745899 ) ;
#89736=VERTEX_POINT ( 'NONE', #94427 ) ;
#89737=EDGE_CURVE ( 'NONE', #92549, #32647, #121062, .T. ) ;
#89738=PLANE ( 'NONE',  #63229 ) ;
#89739=ADVANCED_FACE ( 'NONE', ( #32328 ), #93968, .T. ) ;
#89740=VERTEX_POINT ( 'NONE', #84624 ) ;
#89741=ORIENTED_EDGE ( 'NONE', *, *, #9466, .F. ) ;
#89742=EDGE_CURVE ( 'NONE', #80836, #114385, #106486, .T. ) ;
#89743=CARTESIAN_POINT ( 'NONE',  ( 1.249999999999953815, 2.500000000000000000, 1.472243186433545459 ) ) ;
#89745=LINE ( 'NONE', #29539, #117514 ) ;
#89747=CARTESIAN_POINT ( 'NONE',  ( 0.3999999999999619971, 2.500000000000000000, -0.1000000000000001166 ) ) ;
#89748=AXIS2_PLACEMENT_3D ( 'NONE', #92589, #101119, #52652 ) ;
#89749=EDGE_LOOP ( 'NONE', ( #10872, #18332 ) ) ;
#89750=VERTEX_POINT ( 'NONE', #82706 ) ;
#89751=AXIS2_PLACEMENT_3D ( 'NONE', #32007, #71929, #62108 ) ;
#89752=DIRECTION ( 'NONE',  ( -0.000000000000000000, -1.000000000000000000, -0.000000000000000000 ) ) ;
#89753=VECTOR ( 'NONE', #7158, 1000.000000000000000 ) ;
#89754=ORIENTED_EDGE ( 'NONE', *, *, #20185, .F. ) ;
#89755=DIRECTION ( 'NONE',  ( 0.000000000000000000, 0.000000000000000000, 1.000000000000000000 ) ) ;
#89756=EDGE_LOOP ( 'NONE', ( #113983, #2940, #31599, #19314 ) ) ;
#89757=ORIENTED_EDGE ( 'NONE', *, *, #37211, .T. ) ;
#89758=DIRECTION ( 'NONE',  ( -0.000000000000000000, 1.000000000000000000, -0.000000000000000000 ) ) ;
#89759=CIRCLE ( 'NONE', #41755, 0.09999999999999982514 ) ;
#89760=CARTESIAN_POINT ( 'NONE',  ( 48.81612456492383956, -3.619496399135579523, -4.312668942933988170 ) ) ;
#89761=AXIS2_PLACEMENT_3D ( 'NONE', #69782, #120179, #1674 ) ;
#89762=DIRECTION ( 'NONE',  ( 0.000000000000000000, 0.000000000000000000, 1.000000000000000000 ) ) ;
#89763=CARTESIAN_POINT ( 'NONE',  ( 10.84999999999991260, 12.50000000000000000, -2.857883832488653741 ) ) ;
#89764=DIRECTION ( 'NONE',  ( -0.000000000000000000, 1.000000000000000000, -0.000000000000000000 ) ) ;
#89765=ORIENTED_EDGE ( 'NONE', *, *, #108976, .T. ) ;
#89766=CARTESIAN_POINT ( 'NONE',  ( 6.899999999999926636, 2.500000000000000000, 0.3464101615137736845 ) ) ;
#89767=DIRECTION ( 'NONE',  ( -0.000000000000000000, 1.000000000000000000, -0.000000000000000000 ) ) ;
#89768=DIRECTION ( 'NONE',  ( -0.000000000000000000, -1.000000000000000000, -0.000000000000000000 ) ) ;
#89769=DIRECTION ( 'NONE',  ( 0.000000000000000000, 1.000000000000000000, 0.000000000000000000 ) ) ;
#89770=AXIS2_PLACEMENT_3D ( 'NONE', #115386, #45403, #3532 ) ;
#89771=LINE ( 'NONE', #9285, #20622 ) ;
#89772=ORIENTED_EDGE ( 'NONE', *, *, #35563, .F. ) ;
#89773=AXIS2_PLACEMENT_3D ( 'NONE', #19787, #28317, #19107 ) ;
#89774=EDGE_LOOP ( 'NONE', ( #122777, #62100 ) ) ;
#89775=EDGE_CURVE ( 'NONE', #127091, #39885, #54260, .T. ) ;
#89776=DIRECTION ( 'NONE',  ( 0.000000000000000000, 0.000000000000000000, 1.000000000000000000 ) ) ;
#89777=EDGE_CURVE ( 'NONE', #39666, #86814, #50073, .T. ) ;
#89778=ADVANCED_FACE ( 'NONE', ( #63050 ), #111495, .T. ) ;
#89779=ORIENTED_EDGE ( 'NONE', *, *, #105094, .T. ) ;
#89780=DIRECTION ( 'NONE',  ( 0.000000000000000000, 0.000000000000000000, 1.000000000000000000 ) ) ;
#89781=DIRECTION ( 'NONE',  ( -4.274815082592931898E-19, -0.9999939076577903929, -0.003490651415223739937 ) ) ;
#89782=AXIS2_PLACEMENT_3D ( 'NONE', #62368, #3428, #32274 ) ;
#89783=EDGE_CURVE ( 'NONE', #85004, #46456, #123886, .T. ) ;
#89784=ORIENTED_EDGE ( 'NONE', *, *, #56808, .F. ) ;
#89785=DIRECTION ( 'NONE',  ( -0.000000000000000000, -1.000000000000000000, -0.000000000000000000 ) ) ;
#89786=DIRECTION ( 'NONE',  ( 0.000000000000000000, 0.000000000000000000, -1.000000000000000000 ) ) ;
#89787=EDGE_CURVE ( 'NONE', #102432, #10582, #108627, .T. ) ;
#89788=DIRECTION ( 'NONE',  ( 0.000000000000000000, -0.000000000000000000, 1.000000000000000000 ) ) ;
#89789=DIRECTION ( 'NONE',  ( 0.000000000000000000, -0.000000000000000000, 1.000000000000000000 ) ) ;
#89790=EDGE_CURVE ( 'NONE', #75194, #84422, #122620, .T. ) ;
#89791=ADVANCED_FACE ( 'NONE', ( #72242 ), #45853, .T. ) ;
#89792=EDGE_CURVE ( 'NONE', #65438, #55788, #93168, .T. ) ;
#89793=DIRECTION ( 'NONE',  ( 0.000000000000000000, 0.000000000000000000, 1.000000000000000000 ) ) ;
#89794=ORIENTED_EDGE ( 'NONE', *, *, #45440, .F. ) ;
#89795=CARTESIAN_POINT ( 'NONE',  ( 43.31977652052934502, 2.029676442637600164, -5.113281004118873874 ) ) ;
#89796=CARTESIAN_POINT ( 'NONE',  ( -6.250000000000019540, 12.50000000000000000, -7.122917578226816815 ) ) ;
#89797=ADVANCED_FACE ( 'NONE', ( #51952 ), #110681, .T. ) ;
#89798=DIRECTION ( 'NONE',  ( 0.000000000000000000, 0.000000000000000000, 1.000000000000000000 ) ) ;
#89799=ORIENTED_EDGE ( 'NONE', *, *, #71905, .T. ) ;
#89800=DIRECTION ( 'NONE',  ( 0.000000000000000000, 0.000000000000000000, 1.000000000000000000 ) ) ;
#89801=VERTEX_POINT ( 'NONE', #13935 ) ;
#89802=FACE_OUTER_BOUND ( 'NONE', #59292, .T. ) ;
#89803=CIRCLE ( 'NONE', #68870, 0.06509327318403745899 ) ;
#89804=DIRECTION ( 'NONE',  ( 0.000000000000000000, 0.000000000000000000, 1.000000000000000000 ) ) ;
#89805=DIRECTION ( 'NONE',  ( 0.000000000000000000, 0.000000000000000000, 1.000000000000000000 ) ) ;
#89806=VERTEX_POINT ( 'NONE', #34254 ) ;
#89808=VECTOR ( 'NONE', #24577, 1000.000000000000000 ) ;
#89809=AXIS2_PLACEMENT_3D ( 'NONE', #126201, #57469, #106552 ) ;
#89810=DIRECTION ( 'NONE',  ( 0.000000000000000000, -0.9999939076577903929, 0.003490651415223739937 ) ) ;
#89811=VECTOR ( 'NONE', #36258, 1000.000000000000000 ) ;
#89812=ORIENTED_EDGE ( 'NONE', *, *, #51808, .T. ) ;
#89813=DIRECTION ( 'NONE',  ( -4.274815082592931898E-19, -0.9999939076577903929, -0.003490651415223739937 ) ) ;
#89814=ORIENTED_EDGE ( 'NONE', *, *, #84258, .T. ) ;
#89815=CARTESIAN_POINT ( 'NONE',  ( 13.54999999999989591, 2.500000000000000000, -1.818653347947326138 ) ) ;
#89816=AXIS2_PLACEMENT_3D ( 'NONE', #390, #92013, #99270 ) ;
#89817=CONICAL_SURFACE ( 'NONE', #33413, 0.1000000000000002554, 0.003490658503988666988 ) ;
#89818=VERTEX_POINT ( 'NONE', #112153 ) ;
#89819=DIRECTION ( 'NONE',  ( 0.000000000000000000, 1.000000000000000000, 0.000000000000000000 ) ) ;
#89820=FACE_OUTER_BOUND ( 'NONE', #70609, .T. ) ;
#89821=ORIENTED_EDGE ( 'NONE', *, *, #11878, .F. ) ;
#89822=ORIENTED_EDGE ( 'NONE', *, *, #24041, .T. ) ;
#89823=DIRECTION ( 'NONE',  ( 0.000000000000000000, 0.000000000000000000, 1.000000000000000000 ) ) ;
#89824=DIRECTION ( 'NONE',  ( 0.000000000000000000, 1.000000000000000000, 0.000000000000000000 ) ) ;
#89826=CARTESIAN_POINT ( 'NONE',  ( -0.4000000000000331624, 12.50000000000000000, -0.06509327318403743123 ) ) ;
#89827=CARTESIAN_POINT ( 'NONE',  ( 12.09999999999990195, 12.50000000000000000, -0.6928203230275541413 ) ) ;
#89828=ADVANCED_FACE ( 'NONE', ( #44053 ), #83963, .T. ) ;
#89829=LINE ( 'NONE', #119287, #118457 ) ;
#89831=DIRECTION ( 'NONE',  ( 0.000000000000000000, -0.000000000000000000, 1.000000000000000000 ) ) ;
#89832=LINE ( 'NONE', #111391, #82836 ) ;
#89833=DIRECTION ( 'NONE',  ( 0.000000000000000000, 1.000000000000000000, 0.000000000000000000 ) ) ;
#89834=AXIS2_PLACEMENT_3D ( 'NONE', #121336, #80791, #71597 ) ;
#89835=VECTOR ( 'NONE', #76410, 1000.000000000000000 ) ;
#89836=ORIENTED_EDGE ( 'NONE', *, *, #53226, .F. ) ;
#89838=ORIENTED_EDGE ( 'NONE', *, *, #93664, .T. ) ;
#89839=DIRECTION ( 'NONE',  ( -4.274815082592931898E-19, -0.9999939076577903929, -0.003490651415223739937 ) ) ;
#89840=CARTESIAN_POINT ( 'NONE',  ( 12.89999999999990088, 2.500000000000000000, 4.430127018922196847 ) ) ;
#89841=DIRECTION ( 'NONE',  ( -0.000000000000000000, 1.000000000000000000, -0.000000000000000000 ) ) ;
#89842=VERTEX_POINT ( 'NONE', #121975 ) ;
#89843=FACE_BOUND ( 'NONE', #70853, .T. ) ;
#89844=EDGE_LOOP ( 'NONE', ( #89658, #94473, #7795, #32703 ) ) ;
#89845=CARTESIAN_POINT ( 'NONE',  ( 8.549999999999918998, 2.500000000000000000, -1.918653347947326004 ) ) ;
#89847=CONICAL_SURFACE ( 'NONE', #5918, 0.09999999999999982514, 0.003490658503988666988 ) ;
#89848=AXIS2_PLACEMENT_3D ( 'NONE', #107434, #38055, #7285 ) ;
#89849=CARTESIAN_POINT ( 'NONE',  ( -3.469446951953614189E-14, 12.50000000000000000, -0.6277270498435144619 ) ) ;
#89850=DIRECTION ( 'NONE',  ( -0.000000000000000000, 1.000000000000000000, -0.000000000000000000 ) ) ;
#89851=CARTESIAN_POINT ( 'NONE',  ( -4.550000000000026468, 12.50000000000000000, -6.430097255199264339 ) ) ;
#89852=LINE ( 'NONE', #9368, #45537 ) ;
#89853=FACE_OUTER_BOUND ( 'NONE', #15649, .T. ) ;
#89854=DIRECTION ( 'NONE',  ( 0.000000000000000000, 0.000000000000000000, 1.000000000000000000 ) ) ;
#89855=AXIS2_PLACEMENT_3D ( 'NONE', #80661, #40086, #91756 ) ;
#89856=FACE_OUTER_BOUND ( 'NONE', #43391, .T. ) ;
#89857=VERTEX_POINT ( 'NONE', #92498 ) ;
#89858=VERTEX_POINT ( 'NONE', #54504 ) ;
#89859=AXIS2_PLACEMENT_3D ( 'NONE', #85132, #34773, #125066 ) ;
#89860=ORIENTED_EDGE ( 'NONE', *, *, #60251, .T. ) ;
#89861=VERTEX_POINT ( 'NONE', #91869 ) ;
#89862=DIRECTION ( 'NONE',  ( 0.000000000000000000, -0.000000000000000000, 1.000000000000000000 ) ) ;
#89863=DIRECTION ( 'NONE',  ( 0.000000000000000000, 0.000000000000000000, 1.000000000000000000 ) ) ;
#89865=ORIENTED_EDGE ( 'NONE', *, *, #93955, .T. ) ;
#89866=EDGE_LOOP ( 'NONE', ( #72980, #112761, #65235, #64662 ) ) ;
#89867=CIRCLE ( 'NONE', #4169, 0.09999999999999999167 ) ;
#89868=ORIENTED_EDGE ( 'NONE', *, *, #83785, .F. ) ;
#89869=DIRECTION ( 'NONE',  ( 0.000000000000000000, 0.000000000000000000, 1.000000000000000000 ) ) ;
#89870=CIRCLE ( 'NONE', #77360, 0.1000000000000002554 ) ;
#89871=ADVANCED_FACE ( 'NONE', ( #62421 ), #116931, .T. ) ;
#89872=DIRECTION ( 'NONE',  ( 0.000000000000000000, 1.000000000000000000, 0.000000000000000000 ) ) ;
#89873=DIRECTION ( 'NONE',  ( -0.000000000000000000, -1.000000000000000000, -0.000000000000000000 ) ) ;
#89874=CARTESIAN_POINT ( 'NONE',  ( 12.49999999999990052, 12.50000000000000000, 0.6928203230275494784 ) ) ;
#89875=CARTESIAN_POINT ( 'NONE',  ( -12.49999999999995914, 2.500000000000000000, 1.843143693225357538E-15 ) ) ;
#89876=CIRCLE ( 'NONE', #85751, 0.09999999999999982514 ) ;
#89877=CARTESIAN_POINT ( 'NONE',  ( -3.950000000000028155, 12.50000000000000000, -6.841600689897077814 ) ) ;
#89878=CARTESIAN_POINT ( 'NONE',  ( -5.850000000000021849, 12.50000000000000000, -5.802370205355749988 ) ) ;
#89879=ADVANCED_FACE ( 'NONE', ( #67531 ), #52201, .T. ) ;
#89880=ORIENTED_EDGE ( 'NONE', *, *, #105110, .F. ) ;
#89881=ADVANCED_FACE ( 'NONE', ( #95738 ), #127422, .T. ) ;
#89882=CARTESIAN_POINT ( 'NONE',  ( 0.8499999999999557909, 2.500000000000000000, -7.188010851410854052 ) ) ;
#89883=ORIENTED_EDGE ( 'NONE', *, *, #110080, .T. ) ;
#89884=ORIENTED_EDGE ( 'NONE', *, *, #63929, .T. ) ;
#89885=VERTEX_POINT ( 'NONE', #45997 ) ;
#89886=EDGE_CURVE ( 'NONE', #54425, #18483, #60540, .T. ) ;
#89888=EDGE_CURVE ( 'NONE', #88688, #17050, #77381, .T. ) ;
#89889=ADVANCED_FACE ( 'NONE', ( #115341 ), #75186, .T. ) ;
#89890=ORIENTED_EDGE ( 'NONE', *, *, #106557, .F. ) ;
#89891=EDGE_CURVE ( 'NONE', #54633, #29223, #102294, .T. ) ;
#89892=EDGE_CURVE ( 'NONE', #57396, #110257, #73036, .T. ) ;
#89893=ORIENTED_EDGE ( 'NONE', *, *, #99731, .T. ) ;
#89894=CARTESIAN_POINT ( 'NONE',  ( -3.950000000000024603, 12.50000000000000000, 1.753560074763284016 ) ) ;
#89895=DIRECTION ( 'NONE',  ( 0.000000000000000000, 1.000000000000000000, 0.000000000000000000 ) ) ;
#89896=DIRECTION ( 'NONE',  ( 0.000000000000000000, -0.000000000000000000, 1.000000000000000000 ) ) ;
#89897=CARTESIAN_POINT ( 'NONE',  ( -0.6500000000000398792, 12.50000000000000000, -6.841600689897078702 ) ) ;
#89898=CIRCLE ( 'NONE', #60591, 0.1000000000000002554 ) ;
#89899=ADVANCED_FACE ( 'NONE', ( #85891 ), #36177, .T. ) ;
#89900=ORIENTED_EDGE ( 'NONE', *, *, #110561, .F. ) ;
#89901=DIRECTION ( 'NONE',  ( 0.000000000000000000, 0.000000000000000000, 1.000000000000000000 ) ) ;
#89902=EDGE_CURVE ( 'NONE', #91091, #121671, #66261, .T. ) ;
#89903=VERTEX_POINT ( 'NONE', #75431 ) ;
#89904=DIRECTION ( 'NONE',  ( 0.000000000000000000, 1.000000000000000000, 0.000000000000000000 ) ) ;
#89905=VECTOR ( 'NONE', #65823, 1000.000000000000000 ) ;
#89906=EDGE_LOOP ( 'NONE', ( #51360, #83351 ) ) ;
#89907=CARTESIAN_POINT ( 'NONE',  ( 5.649999999999936406, 2.500000000000000000, -6.841600689897077814 ) ) ;
#89908=DIRECTION ( 'NONE',  ( 0.000000000000000000, 0.000000000000000000, 1.000000000000000000 ) ) ;
#89909=ORIENTED_EDGE ( 'NONE', *, *, #53214, .T. ) ;
#89910=CARTESIAN_POINT ( 'NONE',  ( -10.45000000000000107, 2.500000000000000000, 6.495190528383297135 ) ) ;
#89911=DIRECTION ( 'NONE',  ( -4.274815082592931898E-19, -0.9999939076577903929, -0.003490651415223739937 ) ) ;
#89912=ORIENTED_EDGE ( 'NONE', *, *, #41575, .T. ) ;
#89913=VECTOR ( 'NONE', #125191, 1000.000000000000000 ) ;
#89914=DIRECTION ( 'NONE',  ( 0.000000000000000000, 0.000000000000000000, 1.000000000000000000 ) ) ;
#89915=VERTEX_POINT ( 'NONE', #104886 ) ;
#89916=EDGE_LOOP ( 'NONE', ( #84171, #53204 ) ) ;
#89917=DIRECTION ( 'NONE',  ( 0.000000000000000000, -0.9999939076577903929, 0.003490651415223739937 ) ) ;
#89918=DIRECTION ( 'NONE',  ( -0.000000000000000000, -1.000000000000000000, -0.000000000000000000 ) ) ;
#89920=CARTESIAN_POINT ( 'NONE',  ( 8.299999999999922551, 2.500000000000000000, 4.430127018922196847 ) ) ;
#89922=ORIENTED_EDGE ( 'NONE', *, *, #70197, .F. ) ;
#89923=DIRECTION ( 'NONE',  ( 0.000000000000000000, 0.000000000000000000, 1.000000000000000000 ) ) ;
#89924=ADVANCED_FACE ( 'NONE', ( #125194 ), #31286, .T. ) ;
#89925=ADVANCED_FACE ( 'NONE', ( #117268 ), #87693, .T. ) ;
#89926=VERTEX_POINT ( 'NONE', #124556 ) ;
#89927=FACE_OUTER_BOUND ( 'NONE', #50516, .T. ) ;
#89928=AXIS2_PLACEMENT_3D ( 'NONE', #86991, #28732, #46416 ) ;
#89929=CARTESIAN_POINT ( 'NONE',  ( -7.300000000000014921, 12.50000000000000000, 4.611443907251934426 ) ) ;
#89930=CONICAL_SURFACE ( 'NONE', #23038, 0.1000000000000002554, 0.003490658503988666988 ) ;
#89931=ADVANCED_FACE ( 'NONE', ( #27609 ), #14527, .T. ) ;
#89933=FACE_OUTER_BOUND ( 'NONE', #85907, .T. ) ;
#89934=DIRECTION ( 'NONE',  ( 0.000000000000000000, 1.000000000000000000, 0.000000000000000000 ) ) ;
#89935=EDGE_CURVE ( 'NONE', #21947, #111738, #114718, .T. ) ;
#89936=FACE_OUTER_BOUND ( 'NONE', #75591, .T. ) ;
#89937=LINE ( 'NONE', #88656, #5659 ) ;
#89938=ORIENTED_EDGE ( 'NONE', *, *, #109250, .F. ) ;
#89939=CONICAL_SURFACE ( 'NONE', #25095, 0.1000000000000002554, 0.003490658503988666988 ) ;
#89940=EDGE_CURVE ( 'NONE', #35226, #67849, #68829, .T. ) ;
#89941=LINE ( 'NONE', #111521, #100313 ) ;
#89942=EDGE_CURVE ( 'NONE', #118985, #97598, #91907, .T. ) ;
#89943=DIRECTION ( 'NONE',  ( -0.000000000000000000, 1.000000000000000000, -0.000000000000000000 ) ) ;
#89944=DIRECTION ( 'NONE',  ( 0.000000000000000000, 0.000000000000000000, 1.000000000000000000 ) ) ;
#89945=CIRCLE ( 'NONE', #23061, 0.1000000000000000472 ) ;
#89946=VERTEX_POINT ( 'NONE', #96353 ) ;
#89947=EDGE_CURVE ( 'NONE', #52167, #47194, #89759, .T. ) ;
#89948=CARTESIAN_POINT ( 'NONE',  ( 12.49999999999990585, 2.500000000000000000, -5.022947341949754119 ) ) ;
#89949=CIRCLE ( 'NONE', #52394, 0.06509327318403745899 ) ;
#89950=CONICAL_SURFACE ( 'NONE', #79503, 0.09999999999999982514, 0.003490658503988666988 ) ;
#89951=VERTEX_POINT ( 'NONE', #34899 ) ;
#89952=ORIENTED_EDGE ( 'NONE', *, *, #37051, .F. ) ;
#89953=CARTESIAN_POINT ( 'NONE',  ( 9.799999999999913669, 2.500000000000000000, 4.576537180435972019 ) ) ;
#89954=VERTEX_POINT ( 'NONE', #106819 ) ;
#89955=FACE_OUTER_BOUND ( 'NONE', #71208, .T. ) ;
#89957=CIRCLE ( 'NONE', #31482, 0.06509327318403745899 ) ;
#89958=EDGE_LOOP ( 'NONE', ( #54549, #56632 ) ) ;
#89959=CARTESIAN_POINT ( 'NONE',  ( -3.950000000000025491, 12.50000000000000000, 6.148780366869520897 ) ) ;
#89960=DIRECTION ( 'NONE',  ( 0.000000000000000000, 0.000000000000000000, 1.000000000000000000 ) ) ;
#89961=AXIS2_PLACEMENT_3D ( 'NONE', #46859, #15432, #56643 ) ;
#89962=CARTESIAN_POINT ( 'NONE',  ( -8.150000000000014566, 2.500000000000000000, -6.841600689897073373 ) ) ;
#89963=EDGE_CURVE ( 'NONE', #98405, #99586, #33354, .T. ) ;
#89964=ORIENTED_EDGE ( 'NONE', *, *, #108413, .F. ) ;
#89965=ORIENTED_EDGE ( 'NONE', *, *, #112518, .F. ) ;
#89966=EDGE_LOOP ( 'NONE', ( #23527, #120133 ) ) ;
#89967=FACE_OUTER_BOUND ( 'NONE', #110513, .T. ) ;
#89968=FACE_OUTER_BOUND ( 'NONE', #21739, .T. ) ;
#89969=DIRECTION ( 'NONE',  ( 0.000000000000000000, 0.000000000000000000, 1.000000000000000000 ) ) ;
#89970=FACE_BOUND ( 'NONE', #109182, .T. ) ;
#89971=ORIENTED_EDGE ( 'NONE', *, *, #112669, .T. ) ;
#89972=DIRECTION ( 'NONE',  ( 0.000000000000000000, 0.000000000000000000, 1.000000000000000000 ) ) ;
#89973=CARTESIAN_POINT ( 'NONE',  ( 9.999999999999911182, 12.50000000000000000, -3.572213422710612374 ) ) ;
#89974=ORIENTED_EDGE ( 'NONE', *, *, #33960, .T. ) ;
#89976=CARTESIAN_POINT ( 'NONE',  ( 8.949999999999917577, 2.500000000000000000, 6.048780366869520364 ) ) ;
#89977=EDGE_CURVE ( 'NONE', #123416, #76721, #59033, .T. ) ;
#89978=CIRCLE ( 'NONE', #73262, 0.1000000000000002554 ) ;
#89979=DIRECTION ( 'NONE',  ( 0.000000000000000000, 0.000000000000000000, 1.000000000000000000 ) ) ;
#89980=CARTESIAN_POINT ( 'NONE',  ( 11.44999999999990870, 2.500000000000000000, -1.718653347947326049 ) ) ;
#89981=DIRECTION ( 'NONE',  ( 0.000000000000000000, 1.000000000000000000, 0.000000000000000000 ) ) ;
#89982=CIRCLE ( 'NONE', #39926, 0.06509327318403745899 ) ;
#89983=DIRECTION ( 'NONE',  ( 0.000000000000000000, 0.000000000000000000, 1.000000000000000000 ) ) ;
#89984=CARTESIAN_POINT ( 'NONE',  ( 4.999999999999971578, 2.500000000000000000, -2.276824562219559311E-15 ) ) ;
#89985=VECTOR ( 'NONE', #83975, 1000.000000000000000 ) ;
#89986=EDGE_LOOP ( 'NONE', ( #51018, #63248 ) ) ;
#89987=ORIENTED_EDGE ( 'NONE', *, *, #12305, .F. ) ;
#89988=ORIENTED_EDGE ( 'NONE', *, *, #89004, .F. ) ;
#89989=EDGE_LOOP ( 'NONE', ( #38878, #95275 ) ) ;
#89990=DIRECTION ( 'NONE',  ( 0.000000000000000000, 0.000000000000000000, 1.000000000000000000 ) ) ;
#89991=CARTESIAN_POINT ( 'NONE',  ( 2.499999999999981792, 12.50000000000000000, 4.265033745738159077 ) ) ;
#89993=ADVANCED_FACE ( 'NONE', ( #30235 ), #93780, .T. ) ;
#89994=FACE_BOUND ( 'NONE', #69599, .T. ) ;
#89995=DIRECTION ( 'NONE',  ( 0.000000000000000000, 0.000000000000000000, -1.000000000000000000 ) ) ;
#89996=CARTESIAN_POINT ( 'NONE',  ( 4.349999999999940137, 2.500000000000000000, -6.841600689897078702 ) ) ;
#89997=DIRECTION ( 'NONE',  ( 0.000000000000000000, 0.000000000000000000, 1.000000000000000000 ) ) ;
#89998=DIRECTION ( 'NONE',  ( 0.000000000000000000, 1.000000000000000000, 0.000000000000000000 ) ) ;
#89999=CARTESIAN_POINT ( 'NONE',  ( 12.49999999999990585, 2.500000000000000000, 3.537306695894645081 ) ) ;
#90000=CARTESIAN_POINT ( 'NONE',  ( 5.849999999999932143, 12.50000000000000000, 1.472243186433545459 ) ) ;
#90001=VERTEX_POINT ( 'NONE', #28284 ) ;
#90002=ORIENTED_EDGE ( 'NONE', *, *, #80771, .F. ) ;
#90003=ORIENTED_EDGE ( 'NONE', *, *, #86034, .T. ) ;
#90004=ORIENTED_EDGE ( 'NONE', *, *, #39696, .F. ) ;
#90005=ORIENTED_EDGE ( 'NONE', *, *, #63914, .T. ) ;
#90006=ORIENTED_EDGE ( 'NONE', *, *, #13330, .F. ) ;
#90007=LINE ( 'NONE', #111599, #4562 ) ;
#90008=PLANE ( 'NONE',  #67698 ) ;
#90009=ORIENTED_EDGE ( 'NONE', *, *, #49759, .F. ) ;
#90010=CARTESIAN_POINT ( 'NONE',  ( -9.350000000000004974, 2.500000000000000000, 6.841600689897072485 ) ) ;
#90011=CIRCLE ( 'NONE', #4237, 0.1000000000000000472 ) ;
#90012=ADVANCED_FACE ( 'NONE', ( #98293 ), #112562, .T. ) ;
#90013=DIRECTION ( 'NONE',  ( 0.000000000000000000, 1.000000000000000000, 0.000000000000000000 ) ) ;
#90015=DIRECTION ( 'NONE',  ( 0.000000000000000000, -0.9999939076577903929, 0.003490651415223739937 ) ) ;
#90016=CARTESIAN_POINT ( 'NONE',  ( -13.09999999999999076, 2.500000000000000000, 3.983716857408420964 ) ) ;
#90017=EDGE_LOOP ( 'NONE', ( #58231, #52263 ) ) ;
#90018=FACE_OUTER_BOUND ( 'NONE', #67910, .T. ) ;
#90019=AXIS2_PLACEMENT_3D ( 'NONE', #60041, #111700, #119568 ) ;
#90020=EDGE_CURVE ( 'NONE', #49149, #101786, #18464, .T. ) ;
#90021=VERTEX_POINT ( 'NONE', #48570 ) ;
#90022=VERTEX_POINT ( 'NONE', #99607 ) ;
#90023=FACE_OUTER_BOUND ( 'NONE', #31945, .T. ) ;
#90024=ADVANCED_FACE ( 'NONE', ( #97 ), #35209, .T. ) ;
#90025=DIRECTION ( 'NONE',  ( 0.000000000000000000, -0.000000000000000000, 1.000000000000000000 ) ) ;
#90026=DIRECTION ( 'NONE',  ( 0.000000000000000000, 0.000000000000000000, -1.000000000000000000 ) ) ;
#90027=EDGE_CURVE ( 'NONE', #117051, #88674, #108339, .T. ) ;
#90028=ADVANCED_FACE ( 'NONE', ( #38104 ), #70776, .T. ) ;
#90029=EDGE_CURVE ( 'NONE', #73591, #112590, #128438, .T. ) ;
#90030=EDGE_LOOP ( 'NONE', ( #31862, #48264, #87838, #13478 ) ) ;
#90031=ORIENTED_EDGE ( 'NONE', *, *, #106721, .T. ) ;
#90032=AXIS2_PLACEMENT_3D ( 'NONE', #112499, #31367, #90919 ) ;
#90033=CARTESIAN_POINT ( 'NONE',  ( 4.999999999999938716, 2.500000000000000000, -5.022947341949754119 ) ) ;
#90034=AXIS2_PLACEMENT_3D ( 'NONE', #37184, #18807, #87546 ) ;
#90035=CARTESIAN_POINT ( 'NONE',  ( 4.349999999999937472, 2.500000000000000000, 6.841600689897072485 ) ) ;
#90036=EDGE_CURVE ( 'NONE', #86174, #113061, #10151, .T. ) ;
#90037=CARTESIAN_POINT ( 'NONE',  ( -2.100000000000033840, 2.500000000000000000, 3.537306695894645081 ) ) ;
#90038=ADVANCED_FACE ( 'NONE', ( #19757 ), #89570, .T. ) ;
#90039=CARTESIAN_POINT ( 'NONE',  ( -10.00000000000000355, 12.50000000000000000, 3.637306695894644726 ) ) ;
#90040=EDGE_LOOP ( 'NONE', ( #85248, #87145, #55682, #126605 ) ) ;
#90041=FACE_OUTER_BOUND ( 'NONE', #34573, .T. ) ;
#90042=EDGE_CURVE ( 'NONE', #92801, #101017, #69478, .T. ) ;
#90043=CONICAL_SURFACE ( 'NONE', #92103, 0.1000000000000002554, 0.003490658503988666988 ) ;
#90044=VERTEX_POINT ( 'NONE', #109412 ) ;
#90045=DIRECTION ( 'NONE',  ( 0.000000000000000000, -0.9999939076577903929, 0.003490651415223739937 ) ) ;
#90046=EDGE_CURVE ( 'NONE', #19500, #15955, #89771, .T. ) ;
#90047=EDGE_CURVE ( 'NONE', #110619, #49354, #78017, .T. ) ;
#90048=ORIENTED_EDGE ( 'NONE', *, *, #82460, .T. ) ;
#90049=DIRECTION ( 'NONE',  ( 0.000000000000000000, 0.000000000000000000, 1.000000000000000000 ) ) ;
#90050=DIRECTION ( 'NONE',  ( 0.000000000000000000, 0.000000000000000000, 1.000000000000000000 ) ) ;
#90051=AXIS2_PLACEMENT_3D ( 'NONE', #10756, #8841, #79538 ) ;
#90052=DIRECTION ( 'NONE',  ( 0.000000000000000000, 0.000000000000000000, 1.000000000000000000 ) ) ;
#90053=DIRECTION ( 'NONE',  ( 0.000000000000000000, -0.9999939076577903929, 0.003490651415223739937 ) ) ;
#90054=EDGE_CURVE ( 'NONE', #61247, #30638, #43615, .T. ) ;
#90055=EDGE_LOOP ( 'NONE', ( #80052, #11797, #17178, #75835 ) ) ;
#90056=CARTESIAN_POINT ( 'NONE',  ( 2.699999999999947331, 2.500000000000000000, -0.4464101615137783252 ) ) ;
#90057=DIRECTION ( 'NONE',  ( -0.000000000000000000, 1.000000000000000000, -0.000000000000000000 ) ) ;
#90058=EDGE_LOOP ( 'NONE', ( #31794, #57223, #42922, #44690 ) ) ;
#90059=ORIENTED_EDGE ( 'NONE', *, *, #109915, .F. ) ;
#90060=ORIENTED_EDGE ( 'NONE', *, *, #39277, .T. ) ;
#90061=CARTESIAN_POINT ( 'NONE',  ( -11.84999999999999787, 2.500000000000000000, -6.248780366869523206 ) ) ;
#90062=LINE ( 'NONE', #120829, #76260 ) ;
#90063=CARTESIAN_POINT ( 'NONE',  ( -10.65000000000000213, 2.500000000000000000, 1.818653347947321475 ) ) ;
#90064=FACE_OUTER_BOUND ( 'NONE', #97727, .T. ) ;
#90065=CARTESIAN_POINT ( 'NONE',  ( 6.449999999999930012, 2.500000000000000000, -1.718653347947326049 ) ) ;
#90066=CARTESIAN_POINT ( 'NONE',  ( -6.249999999999984901, 2.500000000000000000, -2.165063509461101710 ) ) ;
#90067=DIRECTION ( 'NONE',  ( 0.000000000000000000, 0.000000000000000000, -1.000000000000000000 ) ) ;
#90068=DIRECTION ( 'NONE',  ( 0.000000000000000000, -0.9999939076577903929, 0.003490651415223739937 ) ) ;
#90069=CARTESIAN_POINT ( 'NONE',  ( -0.2000000000000339284, 12.50000000000000000, -0.3464101615137759604 ) ) ;
#90070=AXIS2_PLACEMENT_3D ( 'NONE', #25171, #65084, #105015 ) ;
#90071=AXIS2_PLACEMENT_3D ( 'NONE', #105538, #55150, #103609 ) ;
#90072=VECTOR ( 'NONE', #41623, 1000.000000000000000 ) ;
#90073=CIRCLE ( 'NONE', #94200, 0.1000000000000002554 ) ;
#90074=VERTEX_POINT ( 'NONE', #40703 ) ;
#90075=CARTESIAN_POINT ( 'NONE',  ( -0.4500000000000402012, 2.500000000000000000, 6.395190528383296602 ) ) ;
#90076=AXIS2_PLACEMENT_3D ( 'NONE', #57366, #13406, #61235 ) ;
#90077=FACE_OUTER_BOUND ( 'NONE', #49834, .T. ) ;
#90078=CARTESIAN_POINT ( 'NONE',  ( -4.800000000000022915, 12.50000000000000000, -0.2813168883297409439 ) ) ;
#90079=DIRECTION ( 'NONE',  ( 0.000000000000000000, 0.000000000000000000, 1.000000000000000000 ) ) ;
#90080=FACE_OUTER_BOUND ( 'NONE', #43094, .T. ) ;
#90081=VERTEX_POINT ( 'NONE', #21030 ) ;
#90082=DIRECTION ( 'NONE',  ( -0.000000000000000000, 1.000000000000000000, -0.000000000000000000 ) ) ;
#90083=EDGE_CURVE ( 'NONE', #127944, #64309, #114596, .T. ) ;
#90084=ADVANCED_FACE ( 'NONE', ( #90399 ), #11200, .T. ) ;
#90085=CARTESIAN_POINT ( 'NONE',  ( 7.899999999999923084, 2.500000000000000000, 0.7928203230275495672 ) ) ;
#90086=DIRECTION ( 'NONE',  ( -0.000000000000000000, -1.000000000000000000, -0.000000000000000000 ) ) ;
#90087=ORIENTED_EDGE ( 'NONE', *, *, #57908, .F. ) ;
#90088=ORIENTED_EDGE ( 'NONE', *, *, #63067, .T. ) ;
#90089=EDGE_CURVE ( 'NONE', #114467, #64833, #56106, .T. ) ;
#90090=CARTESIAN_POINT ( 'NONE',  ( -1.450000000000036371, 12.50000000000000000, 2.511473670974873507 ) ) ;
#90091=TOROIDAL_SURFACE ( 'NONE', #71317, 9.000000000000001776, 1.000000000000000000 ) ;
#90092=ORIENTED_EDGE ( 'NONE', *, *, #53995, .F. ) ;
#90093=ORIENTED_EDGE ( 'NONE', *, *, #90940, .T. ) ;
#90094=DIRECTION ( 'NONE',  ( 0.000000000000000000, 0.000000000000000000, -1.000000000000000000 ) ) ;
#90095=CARTESIAN_POINT ( 'NONE',  ( 18.93069778776544609, 2.571126379696650144, -2.451182541063273490 ) ) ;
#90096=CARTESIAN_POINT ( 'NONE',  ( -4.800000000000026468, 12.50000000000000000, -4.676537180435978769 ) ) ;
#90098=AXIS2_PLACEMENT_3D ( 'NONE', #128261, #57585, #76570 ) ;
#90099=ORIENTED_EDGE ( 'NONE', *, *, #35411, .T. ) ;
#90100=AXIS2_PLACEMENT_3D ( 'NONE', #110969, #80898, #48869 ) ;
#90101=DIRECTION ( 'NONE',  ( 0.000000000000000000, -0.000000000000000000, 1.000000000000000000 ) ) ;
#90102=ORIENTED_EDGE ( 'NONE', *, *, #12413, .T. ) ;
#90103=DIRECTION ( 'NONE',  ( -0.000000000000000000, 1.000000000000000000, -0.000000000000000000 ) ) ;
#90104=CARTESIAN_POINT ( 'NONE',  ( -0.4000000000000339950, 12.50000000000000000, 0.6277270498435143509 ) ) ;
#90105=DIRECTION ( 'NONE',  ( -0.000000000000000000, -1.000000000000000000, -0.000000000000000000 ) ) ;
#90106=AXIS2_PLACEMENT_3D ( 'NONE', #89897, #10671, #11981 ) ;
#90107=EDGE_LOOP ( 'NONE', ( #105001, #53281, #95330, #121211 ) ) ;
#90108=AXIS2_PLACEMENT_3D ( 'NONE', #31475, #72690, #112616 ) ;
#90109=ORIENTED_EDGE ( 'NONE', *, *, #99350, .T. ) ;
#90110=ORIENTED_EDGE ( 'NONE', *, *, #90831, .T. ) ;
#90111=ORIENTED_EDGE ( 'NONE', *, *, #64807, .T. ) ;
#90112=ORIENTED_EDGE ( 'NONE', *, *, #78593, .T. ) ;
#90113=CARTESIAN_POINT ( 'NONE',  ( 0.8499999999999527933, 2.500000000000000000, 7.088010851410848190 ) ) ;
#90114=CARTESIAN_POINT ( 'NONE',  ( 15.50668944026764962, 2.500000000000127010, 6.997696164093728299 ) ) ;
#90115=CARTESIAN_POINT ( 'NONE',  ( 12.94999999999989981, 2.500000000000000000, -2.065063509461102065 ) ) ;
#90116=FACE_BOUND ( 'NONE', #81974, .T. ) ;
#90117=CARTESIAN_POINT ( 'NONE',  ( -8.150000000000012790, 12.50000000000000000, -2.446380397790840266 ) ) ;
#90119=CARTESIAN_POINT ( 'NONE',  ( 12.29999999999990479, 12.50000000000000000, 4.676537180435972552 ) ) ;
#90120=CARTESIAN_POINT ( 'NONE',  ( -2.950000000000033484, 12.50000000000000000, -6.495190528383302464 ) ) ;
#90121=AXIS2_PLACEMENT_3D ( 'NONE', #125524, #105243, #124251 ) ;
#90122=CONICAL_SURFACE ( 'NONE', #2380, 0.09999999999999982514, 0.003490658503988666988 ) ;
#90123=DIRECTION ( 'NONE',  ( 0.000000000000000000, 1.000000000000000000, 0.000000000000000000 ) ) ;
#90124=FACE_OUTER_BOUND ( 'NONE', #105611, .T. ) ;
#90125=LINE ( 'NONE', #77730, #126466 ) ;
#90126=CIRCLE ( 'NONE', #94337, 0.06509327318403745899 ) ;
#90127=DIRECTION ( 'NONE',  ( 0.000000000000000000, 0.000000000000000000, 1.000000000000000000 ) ) ;
#90128=ORIENTED_EDGE ( 'NONE', *, *, #29388, .T. ) ;
#90129=CONICAL_SURFACE ( 'NONE', #50351, 0.09999999999999982514, 0.003490658503988666988 ) ;
#90130=CIRCLE ( 'NONE', #39999, 0.09999999999999999167 ) ;
#90131=EDGE_LOOP ( 'NONE', ( #11338, #18577, #113282, #12854 ) ) ;
#90132=ORIENTED_EDGE ( 'NONE', *, *, #51155, .T. ) ;
#90133=ORIENTED_EDGE ( 'NONE', *, *, #67126, .F. ) ;
#90134=EDGE_CURVE ( 'NONE', #3310, #24288, #45668, .T. ) ;
#90135=CARTESIAN_POINT ( 'NONE',  ( 8.349999999999919709, 12.50000000000000000, -2.922977105672691422 ) ) ;
#90136=DIRECTION ( 'NONE',  ( 0.000000000000000000, 1.000000000000000000, 0.000000000000000000 ) ) ;
#90137=EDGE_CURVE ( 'NONE', #86700, #108664, #6207, .T. ) ;
#90138=FACE_BOUND ( 'NONE', #89906, .T. ) ;
#90139=DIRECTION ( 'NONE',  ( -4.274815082592931898E-19, -0.9999939076577903929, -0.003490651415223739937 ) ) ;
#90140=ORIENTED_EDGE ( 'NONE', *, *, #71847, .T. ) ;
#90141=DIRECTION ( 'NONE',  ( -4.274815082592931898E-19, -0.9999939076577903929, -0.003490651415223739937 ) ) ;
#90142=CARTESIAN_POINT ( 'NONE',  ( 14.14999999999989200, 2.500000000000000000, -2.165063509461101710 ) ) ;
#90143=EDGE_CURVE ( 'NONE', #10563, #62105, #1726, .T. ) ;
#90144=DIRECTION ( 'NONE',  ( -0.000000000000000000, 1.000000000000000000, -0.000000000000000000 ) ) ;
#90145=CARTESIAN_POINT ( 'NONE',  ( -2.100000000000033396, 12.50000000000000000, -5.088040615133791356 ) ) ;
#90146=ORIENTED_EDGE ( 'NONE', *, *, #73747, .T. ) ;
#90147=FACE_OUTER_BOUND ( 'NONE', #33035, .T. ) ;
#90148=EDGE_LOOP ( 'NONE', ( #127599, #57978 ) ) ;
#90150=VECTOR ( 'NONE', #66883, 1000.000000000000000 ) ;
#90151=CARTESIAN_POINT ( 'NONE',  ( -5.600000000000023626, 12.50000000000000000, -4.676537180435977881 ) ) ;
#90153=ORIENTED_EDGE ( 'NONE', *, *, #45037, .F. ) ;
#90154=DIRECTION ( 'NONE',  ( 0.000000000000000000, 0.000000000000000000, 1.000000000000000000 ) ) ;
#90155=AXIS2_PLACEMENT_3D ( 'NONE', #92353, #114569, #107981 ) ;
#90156=CARTESIAN_POINT ( 'NONE',  ( 8.949999999999919353, 12.50000000000000000, -6.148780366869526226 ) ) ;
#90157=AXIS2_PLACEMENT_3D ( 'NONE', #5016, #44971, #84877 ) ;
#90158=ADVANCED_FACE ( 'NONE', ( #92338 ), #129305, .T. ) ;
#90159=DIRECTION ( 'NONE',  ( 0.000000000000000000, 0.000000000000000000, -1.000000000000000000 ) ) ;
#90160=VERTEX_POINT ( 'NONE', #62894 ) ;
#90161=AXIS2_PLACEMENT_3D ( 'NONE', #118057, #126607, #36934 ) ;
#90162=DIRECTION ( 'NONE',  ( 0.000000000000000000, 1.000000000000000000, 0.000000000000000000 ) ) ;
#90163=VERTEX_POINT ( 'NONE', #121166 ) ;
#90164=DIRECTION ( 'NONE',  ( -0.000000000000000000, -1.000000000000000000, -0.000000000000000000 ) ) ;
#90165=EDGE_CURVE ( 'NONE', #93275, #122496, #60344, .T. ) ;
#90166=ORIENTED_EDGE ( 'NONE', *, *, #66849, .T. ) ;
#90168=ORIENTED_EDGE ( 'NONE', *, *, #24921, .F. ) ;
#90169=DIRECTION ( 'NONE',  ( -0.000000000000000000, -1.000000000000000000, -0.000000000000000000 ) ) ;
#90170=DIRECTION ( 'NONE',  ( 0.000000000000000000, 1.000000000000000000, 0.000000000000000000 ) ) ;
#90171=EDGE_CURVE ( 'NONE', #66106, #79633, #106294, .T. ) ;
#90172=CARTESIAN_POINT ( 'NONE',  ( 1.449999999999951328, 12.50000000000000000, 2.576566944158910744 ) ) ;
#90173=FACE_OUTER_BOUND ( 'NONE', #122726, .T. ) ;
#90174=EDGE_CURVE ( 'NONE', #57536, #67817, #95834, .T. ) ;
#90175=ADVANCED_FACE ( 'NONE', ( #93645 ), #83325, .T. ) ;
#90176=CARTESIAN_POINT ( 'NONE',  ( 3.549999999999943867, 12.50000000000000000, -6.083687093685488989 ) ) ;
#90177=EDGE_CURVE ( 'NONE', #56615, #118548, #3878, .T. ) ;
#90178=EDGE_LOOP ( 'NONE', ( #38981, #43881, #33461, #28649 ) ) ;
#90179=VERTEX_POINT ( 'NONE', #41970 ) ;
#90180=ORIENTED_EDGE ( 'NONE', *, *, #120813, .F. ) ;
#90181=CARTESIAN_POINT ( 'NONE',  ( -0.8500000000000390576, 12.50000000000000000, -2.165063509461101710 ) ) ;
#90182=LINE ( 'NONE', #40486, #43149 ) ;
#90183=ADVANCED_FACE ( 'NONE', ( #64175 ), #26874, .T. ) ;
#90184=LINE ( 'NONE', #98090, #35539 ) ;
#90186=ORIENTED_EDGE ( 'NONE', *, *, #28265, .F. ) ;
#90188=EDGE_CURVE ( 'NONE', #125479, #19146, #68919, .T. ) ;
#90189=CARTESIAN_POINT ( 'NONE',  ( 4.149999999999938183, 12.50000000000000000, 5.867463478539781896 ) ) ;
#90190=AXIS2_PLACEMENT_3D ( 'NONE', #118261, #66580, #6349 ) ;
#90191=EDGE_LOOP ( 'NONE', ( #29189, #94212, #17120, #21767 ) ) ;
#90192=CARTESIAN_POINT ( 'NONE',  ( 4.399999999999939071, 2.500000000000000000, 0.2464101615137736789 ) ) ;
#90193=AXIS2_PLACEMENT_3D ( 'NONE', #28420, #58533, #98421 ) ;
#90194=EDGE_CURVE ( 'NONE', #47712, #13125, #77051, .T. ) ;
#90195=CARTESIAN_POINT ( 'NONE',  ( -3.950000000000026379, 2.500000000000000000, 2.511473670974873507 ) ) ;
#90196=LINE ( 'NONE', #40501, #102462 ) ;
#90197=DIRECTION ( 'NONE',  ( -4.274815082592931898E-19, -0.9999939076577903929, -0.003490651415223739937 ) ) ;
#90198=CARTESIAN_POINT ( 'NONE',  ( -7.900000000000014566, 2.500000000000000000, 0.09999999999999772959 ) ) ;
#90199=DIRECTION ( 'NONE',  ( 0.000000000000000000, 0.000000000000000000, 1.000000000000000000 ) ) ;
#90200=EDGE_CURVE ( 'NONE', #30524, #20308, #97875, .T. ) ;
#90201=PLANE ( 'NONE',  #102202 ) ;
#90202=AXIS2_PLACEMENT_3D ( 'NONE', #92875, #32683, #12359 ) ;
#90203=ADVANCED_FACE ( 'NONE', ( #81869 ), #12482, .T. ) ;
#90204=VERTEX_POINT ( 'NONE', #74002 ) ;
#90205=ORIENTED_EDGE ( 'NONE', *, *, #106943, .T. ) ;
#90206=DIRECTION ( 'NONE',  ( 0.000000000000000000, 0.000000000000000000, -1.000000000000000000 ) ) ;
#90207=AXIS2_PLACEMENT_3D ( 'NONE', #17467, #67866, #107801 ) ;
#90208=DIRECTION ( 'NONE',  ( 0.000000000000000000, 1.000000000000000000, 0.000000000000000000 ) ) ;
#90209=ORIENTED_EDGE ( 'NONE', *, *, #47915, .T. ) ;
#90210=VERTEX_POINT ( 'NONE', #83189 ) ;
#90212=CARTESIAN_POINT ( 'NONE',  ( 7.299999999999926104, 12.50000000000000000, -0.3464101615137782364 ) ) ;
#90213=DIRECTION ( 'NONE',  ( 0.000000000000000000, 0.000000000000000000, -1.000000000000000000 ) ) ;
#90214=AXIS2_PLACEMENT_3D ( 'NONE', #85445, #36373, #76278 ) ;
#90215=DIRECTION ( 'NONE',  ( -0.000000000000000000, 1.000000000000000000, -0.000000000000000000 ) ) ;
#90217=AXIS2_PLACEMENT_3D ( 'NONE', #76139, #18501, #28985 ) ;
#90218=FACE_OUTER_BOUND ( 'NONE', #6684, .T. ) ;
#90219=FACE_OUTER_BOUND ( 'NONE', #74359, .T. ) ;
#90220=AXIS2_PLACEMENT_3D ( 'NONE', #18777, #48908, #88812 ) ;
#90221=DIRECTION ( 'NONE',  ( 0.000000000000000000, 1.000000000000000000, 0.000000000000000000 ) ) ;
#90222=AXIS2_PLACEMENT_3D ( 'NONE', #52626, #12057, #2895 ) ;
#90223=CARTESIAN_POINT ( 'NONE',  ( 4.599999999999938360, 2.500000000000000000, -0.1000000000000022815 ) ) ;
#90224=ORIENTED_EDGE ( 'NONE', *, *, #6556, .T. ) ;
#90225=ORIENTED_EDGE ( 'NONE', *, *, #118392, .T. ) ;
#90226=VECTOR ( 'NONE', #38164, 1000.000000000000000 ) ;
#90227=AXIS2_PLACEMENT_3D ( 'NONE', #99257, #29229, #100519 ) ;
#90228=ORIENTED_EDGE ( 'NONE', *, *, #99090, .T. ) ;
#90229=ORIENTED_EDGE ( 'NONE', *, *, #108089, .T. ) ;
#90230=ORIENTED_EDGE ( 'NONE', *, *, #1976, .T. ) ;
#90231=DIRECTION ( 'NONE',  ( 0.000000000000000000, 1.000000000000000000, 0.000000000000000000 ) ) ;
#90232=DIRECTION ( 'NONE',  ( 0.000000000000000000, 1.000000000000000000, 0.000000000000000000 ) ) ;
#90233=EDGE_LOOP ( 'NONE', ( #59841, #55484 ) ) ;
#90234=LINE ( 'NONE', #88301, #100906 ) ;
#90235=EDGE_CURVE ( 'NONE', #68041, #91784, #41480, .T. ) ;
#90236=CARTESIAN_POINT ( 'NONE',  ( 10.64999999999990976, 2.500000000000000000, -6.941600689897077459 ) ) ;
#90238=DIRECTION ( 'NONE',  ( 0.000000000000000000, 1.000000000000000000, 0.000000000000000000 ) ) ;
#90239=DIRECTION ( 'NONE',  ( -0.000000000000000000, -1.000000000000000000, -0.000000000000000000 ) ) ;
#90240=ORIENTED_EDGE ( 'NONE', *, *, #86029, .F. ) ;
#90241=LINE ( 'NONE', #121646, #74632 ) ;
#90242=CARTESIAN_POINT ( 'NONE',  ( 8.749999999999920064, 12.50000000000000000, 5.737276932171707422 ) ) ;
#90244=ORIENTED_EDGE ( 'NONE', *, *, #114298, .T. ) ;
#90245=EDGE_LOOP ( 'NONE', ( #122247, #45201, #14806, #53968 ) ) ;
#90246=AXIS2_PLACEMENT_3D ( 'NONE', #79206, #96887, #98822 ) ;
#90247=ORIENTED_EDGE ( 'NONE', *, *, #74581, .T. ) ;
#90248=DIRECTION ( 'NONE',  ( 0.000000000000000000, 1.000000000000000000, 0.000000000000000000 ) ) ;
#90249=VECTOR ( 'NONE', #100542, 1000.000000000000000 ) ;
#90250=CARTESIAN_POINT ( 'NONE',  ( -7.950000000000012612, 12.50000000000000000, 2.230156782645134950 ) ) ;
#90251=DIRECTION ( 'NONE',  ( 0.000000000000000000, 1.000000000000000000, 0.000000000000000000 ) ) ;
#90252=AXIS2_PLACEMENT_3D ( 'NONE', #14284, #32027, #52940 ) ;
#90253=CIRCLE ( 'NONE', #104922, 0.06509327318403745899 ) ;
#90254=DIRECTION ( 'NONE',  ( 0.000000000000000000, 0.000000000000000000, -1.000000000000000000 ) ) ;
#90255=VECTOR ( 'NONE', #33063, 1000.000000000000000 ) ;
#90256=ORIENTED_EDGE ( 'NONE', *, *, #33951, .T. ) ;
#90257=FACE_OUTER_BOUND ( 'NONE', #9786, .T. ) ;
#90258=DIRECTION ( 'NONE',  ( -0.000000000000000000, 1.000000000000000000, -0.000000000000000000 ) ) ;
#90259=CIRCLE ( 'NONE', #84005, 0.1000000000000000472 ) ;
#90260=DIRECTION ( 'NONE',  ( -0.000000000000000000, 1.000000000000000000, -0.000000000000000000 ) ) ;
#90261=CARTESIAN_POINT ( 'NONE',  ( 1.249999999999988454, 2.500000000000000000, 2.165063509461097713 ) ) ;
#90262=CIRCLE ( 'NONE', #106992, 0.06509327318403745899 ) ;
#90263=VERTEX_POINT ( 'NONE', #124398 ) ;
#90264=DIRECTION ( 'NONE',  ( -4.274815082592931898E-19, -0.9999939076577903929, -0.003490651415223739937 ) ) ;
#90265=ORIENTED_EDGE ( 'NONE', *, *, #72595, .F. ) ;
#90266=ORIENTED_EDGE ( 'NONE', *, *, #125597, .T. ) ;
#90267=DIRECTION ( 'NONE',  ( -0.000000000000000000, -1.000000000000000000, -0.000000000000000000 ) ) ;
#90268=CARTESIAN_POINT ( 'NONE',  ( 9.149999999999915090, 12.50000000000000000, 6.495190528383297135 ) ) ;
#90269=FACE_BOUND ( 'NONE', #110156, .T. ) ;
#90270=FACE_OUTER_BOUND ( 'NONE', #123865, .T. ) ;
#90271=CARTESIAN_POINT ( 'NONE',  ( 3.949999999999942446, 2.500000000000000000, -6.841600689897078702 ) ) ;
#90272=CARTESIAN_POINT ( 'NONE',  ( -2.900000000000030109, 12.50000000000000000, -3.637306695894650055 ) ) ;
#90273=EDGE_CURVE ( 'NONE', #29184, #43211, #76582, .T. ) ;
#90274=FACE_OUTER_BOUND ( 'NONE', #52408, .T. ) ;
#90275=FACE_OUTER_BOUND ( 'NONE', #103173, .T. ) ;
#90276=CARTESIAN_POINT ( 'NONE',  ( 5.599999999999931255, 2.500000000000000000, 4.083716857408420609 ) ) ;
#90277=CARTESIAN_POINT ( 'NONE',  ( -6.650000000000018119, 2.500000000000000000, -2.065063509461102065 ) ) ;
#90278=VERTEX_POINT ( 'NONE', #56281 ) ;
#90279=VECTOR ( 'NONE', #21350, 1000.000000000000000 ) ;
#90280=DIRECTION ( 'NONE',  ( 0.000000000000000000, -0.000000000000000000, 1.000000000000000000 ) ) ;
#90281=AXIS2_PLACEMENT_3D ( 'NONE', #48548, #49211, #117916 ) ;
#90282=PLANE ( 'NONE',  #3639 ) ;
#90283=ORIENTED_EDGE ( 'NONE', *, *, #82078, .T. ) ;
#90284=ORIENTED_EDGE ( 'NONE', *, *, #84585, .T. ) ;
#90285=EDGE_CURVE ( 'NONE', #116013, #109874, #26193, .T. ) ;
#90286=DIRECTION ( 'NONE',  ( 0.000000000000000000, -0.000000000000000000, 1.000000000000000000 ) ) ;
#90287=CARTESIAN_POINT ( 'NONE',  ( 9.149999999999920419, 12.50000000000000000, 2.792790559304612064 ) ) ;
#90288=ADVANCED_FACE ( 'NONE', ( #105395 ), #10243, .T. ) ;
#90289=FACE_BOUND ( 'NONE', #76217, .T. ) ;
#90290=AXIS2_PLACEMENT_3D ( 'NONE', #35245, #46994, #86898 ) ;
#90291=CARTESIAN_POINT ( 'NONE',  ( 6.449999999999930012, 12.50000000000000000, -1.818653347947326138 ) ) ;
#90292=CONICAL_SURFACE ( 'NONE', #65152, 0.09999999999999999167, 0.003490658503988666988 ) ;
#90293=AXIS2_PLACEMENT_3D ( 'NONE', #108107, #50479, #110051 ) ;
#90294=AXIS2_PLACEMENT_3D ( 'NONE', #16508, #36184, #76740 ) ;
#90295=FACE_OUTER_BOUND ( 'NONE', #24831, .T. ) ;
#90297=EDGE_LOOP ( 'NONE', ( #120847, #72205 ) ) ;
#90298=FACE_OUTER_BOUND ( 'NONE', #12705, .T. ) ;
#90300=DIRECTION ( 'NONE',  ( -0.000000000000000000, 1.000000000000000000, -0.000000000000000000 ) ) ;
#90301=EDGE_LOOP ( 'NONE', ( #2661, #102463, #32885, #82076 ) ) ;
#90302=AXIS2_PLACEMENT_3D ( 'NONE', #15069, #26863, #45869 ) ;
#90303=CARTESIAN_POINT ( 'NONE',  ( 5.799999999999933209, 12.50000000000000000, -2.385244779468109755E-15 ) ) ;
#90304=DIRECTION ( 'NONE',  ( 0.000000000000000000, 1.000000000000000000, 0.000000000000000000 ) ) ;
#90305=AXIS2_PLACEMENT_3D ( 'NONE', #1436, #119933, #135 ) ;
#90306=CONICAL_SURFACE ( 'NONE', #67307, 0.1000000000000002554, 0.003490658503988666988 ) ;
#90307=CONICAL_SURFACE ( 'NONE', #36048, 0.09999999999999999167, 0.003490658503988666988 ) ;
#90308=CARTESIAN_POINT ( 'NONE',  ( 6.649999999999928413, 2.500000000000000000, 2.757883832488649656 ) ) ;
#90309=FACE_OUTER_BOUND ( 'NONE', #32992, .T. ) ;
#90310=ORIENTED_EDGE ( 'NONE', *, *, #10260, .T. ) ;
#90311=CARTESIAN_POINT ( 'NONE',  ( 12.09999999999990550, 2.500000000000000000, 5.122947341949749323 ) ) ;
#90312=CIRCLE ( 'NONE', #88158, 0.06509327318403745899 ) ;
#90313=DIRECTION ( 'NONE',  ( -0.000000000000000000, 1.000000000000000000, -0.000000000000000000 ) ) ;
#90314=DIRECTION ( 'NONE',  ( 0.000000000000000000, 0.000000000000000000, 1.000000000000000000 ) ) ;
#90315=CARTESIAN_POINT ( 'NONE',  ( -7.050000000000013145, 12.50000000000000000, 6.495190528383297135 ) ) ;
#90316=ORIENTED_EDGE ( 'NONE', *, *, #37731, .T. ) ;
#90317=ORIENTED_EDGE ( 'NONE', *, *, #112530, .F. ) ;
#90318=DIRECTION ( 'NONE',  ( 0.000000000000000000, 1.000000000000000000, 0.000000000000000000 ) ) ;
#90319=EDGE_LOOP ( 'NONE', ( #30117, #74752 ) ) ;
#90320=DIRECTION ( 'NONE',  ( -0.000000000000000000, -1.000000000000000000, -0.000000000000000000 ) ) ;
#90321=CARTESIAN_POINT ( 'NONE',  ( 3.949999999999938005, 2.500000000000000000, 6.841600689897072485 ) ) ;
#90322=EDGE_CURVE ( 'NONE', #32289, #11740, #5880, .T. ) ;
#90323=DIRECTION ( 'NONE',  ( 0.000000000000000000, 1.000000000000000000, 0.000000000000000000 ) ) ;
#90324=ORIENTED_EDGE ( 'NONE', *, *, #12912, .T. ) ;
#90325=DIRECTION ( 'NONE',  ( -4.274815082592931898E-19, -0.9999939076577903929, -0.003490651415223739937 ) ) ;
#90326=DIRECTION ( 'NONE',  ( 0.000000000000000000, 0.000000000000000000, -1.000000000000000000 ) ) ;
#90327=CARTESIAN_POINT ( 'NONE',  ( -12.09999999999999432, 2.500000000000000000, 5.022947341949748790 ) ) ;
#90328=LINE ( 'NONE', #119812, #20395 ) ;
#90329=DIRECTION ( 'NONE',  ( 0.000000000000000000, 0.000000000000000000, 1.000000000000000000 ) ) ;
#90330=ADVANCED_FACE ( 'NONE', ( #64815 ), #67362, .T. ) ;
#90331=CARTESIAN_POINT ( 'NONE',  ( 0.5999999999999612310, 12.50000000000000000, -0.3464101615137760715 ) ) ;
#90332=ADVANCED_FACE ( 'NONE', ( #114556 ), #95917, .T. ) ;
#90333=ORIENTED_EDGE ( 'NONE', *, *, #88631, .F. ) ;
#90334=EDGE_LOOP ( 'NONE', ( #51783, #114739 ) ) ;
#90335=CARTESIAN_POINT ( 'NONE',  ( -11.24999999999996270, 2.500000000000000000, 6.495190528383297135 ) ) ;
#90336=VERTEX_POINT ( 'NONE', #16965 ) ;
#90337=AXIS2_PLACEMENT_3D ( 'NONE', #80975, #31240, #111047 ) ;
#90338=CARTESIAN_POINT ( 'NONE',  ( -4.150000000000025224, 2.500000000000000000, 7.188010851410848723 ) ) ;
#90339=CIRCLE ( 'NONE', #84088, 0.1000000000000002554 ) ;
#90340=EDGE_CURVE ( 'NONE', #24778, #44661, #6021, .T. ) ;
#90341=CIRCLE ( 'NONE', #125852, 0.09999999999999982514 ) ;
#90342=ORIENTED_EDGE ( 'NONE', *, *, #36321, .F. ) ;
#90343=ORIENTED_EDGE ( 'NONE', *, *, #36901, .F. ) ;
#90344=EDGE_CURVE ( 'NONE', #99703, #93625, #125028, .T. ) ;
#90345=ORIENTED_EDGE ( 'NONE', *, *, #115428, .T. ) ;
#90346=EDGE_CURVE ( 'NONE', #111372, #65580, #84467, .T. ) ;
#90347=CARTESIAN_POINT ( 'NONE',  ( 17.50000000000000000, 1.666666666666669627, -3.999999999999996447 ) ) ;
#90348=EDGE_CURVE ( 'NONE', #28873, #49975, #89665, .T. ) ;
#90349=PLANE ( 'NONE',  #84096 ) ;
#90350=AXIS2_PLACEMENT_3D ( 'NONE', #94793, #107177, #85611 ) ;
#90351=CONICAL_SURFACE ( 'NONE', #125859, 0.1000000000000000472, 0.003490658503988666988 ) ;
#90352=CARTESIAN_POINT ( 'NONE',  ( 7.949999999999925571, 12.50000000000000000, 2.165063509461097713 ) ) ;
#90353=VECTOR ( 'NONE', #58349, 1000.000000000000000 ) ;
#90354=EDGE_CURVE ( 'NONE', #4982, #56070, #24816, .T. ) ;
#90355=CARTESIAN_POINT ( 'NONE',  ( -3.150000000000033218, 2.500000000000000000, -6.741600689897078169 ) ) ;
#90356=DIRECTION ( 'NONE',  ( 0.000000000000000000, -0.9999939076577903929, 0.003490651415223739937 ) ) ;
#90357=DIRECTION ( 'NONE',  ( 0.000000000000000000, -0.9999939076577903929, 0.003490651415223739937 ) ) ;
#90358=DIRECTION ( 'NONE',  ( -0.000000000000000000, 1.000000000000000000, -0.000000000000000000 ) ) ;
#90359=DIRECTION ( 'NONE',  ( 0.000000000000000000, 0.000000000000000000, -1.000000000000000000 ) ) ;
#90361=DIRECTION ( 'NONE',  ( -0.000000000000000000, 1.000000000000000000, -0.000000000000000000 ) ) ;
#90362=EDGE_CURVE ( 'NONE', #35098, #73050, #97969, .T. ) ;
#90363=AXIS2_PLACEMENT_3D ( 'NONE', #24079, #63999, #105204 ) ;
#90364=ORIENTED_EDGE ( 'NONE', *, *, #28221, .F. ) ;
#90365=FACE_OUTER_BOUND ( 'NONE', #2450, .T. ) ;
#90367=ORIENTED_EDGE ( 'NONE', *, *, #29686, .F. ) ;
#90368=FACE_OUTER_BOUND ( 'NONE', #87053, .T. ) ;
#90369=FACE_OUTER_BOUND ( 'NONE', #26272, .T. ) ;
#90370=DIRECTION ( 'NONE',  ( 0.000000000000000000, 0.000000000000000000, -1.000000000000000000 ) ) ;
#90371=CARTESIAN_POINT ( 'NONE',  ( -9.600000000000006750, 2.500000000000000000, 0.6928203230275494784 ) ) ;
#90372=CARTESIAN_POINT ( 'NONE',  ( -12.04999999999999538, 12.50000000000000000, 6.495190528383297135 ) ) ;
#90373=DIRECTION ( 'NONE',  ( -0.000000000000000000, -1.000000000000000000, -0.000000000000000000 ) ) ;
#90374=EDGE_LOOP ( 'NONE', ( #118746, #26338, #39377, #15083 ) ) ;
#90375=AXIS2_PLACEMENT_3D ( 'NONE', #39587, #41515, #109593 ) ;
#90376=EDGE_LOOP ( 'NONE', ( #24326, #81706 ) ) ;
#90377=CARTESIAN_POINT ( 'NONE',  ( -4.600000000000028066, 2.500000000000000000, -3.737306695894649700 ) ) ;
#90378=ORIENTED_EDGE ( 'NONE', *, *, #105742, .T. ) ;
#90379=DIRECTION ( 'NONE',  ( 0.000000000000000000, 0.000000000000000000, 1.000000000000000000 ) ) ;
#90380=ORIENTED_EDGE ( 'NONE', *, *, #54044, .T. ) ;
#90381=EDGE_LOOP ( 'NONE', ( #57452, #55267, #72853, #34040 ) ) ;
#90382=AXIS2_PLACEMENT_3D ( 'NONE', #56621, #86076, #73693 ) ;
#90383=DIRECTION ( 'NONE',  ( -0.000000000000000000, 1.000000000000000000, -0.000000000000000000 ) ) ;
#90384=CARTESIAN_POINT ( 'NONE',  ( 65.38811649227264411, -3.824344232458583459, -5.305600839591994244 ) ) ;
#90385=VECTOR ( 'NONE', #90533, 1000.000000000000000 ) ;
#90386=AXIS2_PLACEMENT_3D ( 'NONE', #10013, #100332, #49962 ) ;
#90387=DIRECTION ( 'NONE',  ( 0.000000000000000000, 1.000000000000000000, 0.000000000000000000 ) ) ;
#90388=AXIS2_PLACEMENT_3D ( 'NONE', #8139, #97816, #48087 ) ;
#90389=EDGE_CURVE ( 'NONE', #30036, #75419, #35294, .T. ) ;
#90390=CARTESIAN_POINT ( 'NONE',  ( 2.099999999999949463, 12.50000000000000000, 0.6928203230275494784 ) ) ;
#90391=CARTESIAN_POINT ( 'NONE',  ( 87.50000000000001421, 3.413194297214861894, 6.711110875543778498 ) ) ;
#90392=ORIENTED_EDGE ( 'NONE', *, *, #16438, .F. ) ;
#90393=CARTESIAN_POINT ( 'NONE',  ( -3.150000000000032330, 2.500000000000000000, -6.148780366869526226 ) ) ;
#90394=DIRECTION ( 'NONE',  ( 0.000000000000000000, 1.000000000000000000, 0.000000000000000000 ) ) ;
#90395=CARTESIAN_POINT ( 'NONE',  ( 5.199999999999935341, 2.500000000000000000, -0.3464101615137783474 ) ) ;
#90396=DIRECTION ( 'NONE',  ( 0.000000000000000000, 0.000000000000000000, 1.000000000000000000 ) ) ;
#90397=AXIS2_PLACEMENT_3D ( 'NONE', #107993, #79826, #9154 ) ;
#90398=AXIS2_PLACEMENT_3D ( 'NONE', #37991, #26249, #58294 ) ;
#90399=FACE_OUTER_BOUND ( 'NONE', #27714, .T. ) ;
#90400=EDGE_CURVE ( 'NONE', #56590, #95073, #54997, .T. ) ;
#90401=ORIENTED_EDGE ( 'NONE', *, *, #82820, .T. ) ;
#90402=AXIS2_PLACEMENT_3D ( 'NONE', #116444, #26788, #35967 ) ;
#90403=AXIS2_PLACEMENT_3D ( 'NONE', #5204, #43238, #102763 ) ;
#90404=ORIENTED_EDGE ( 'NONE', *, *, #98833, .T. ) ;
#90405=CARTESIAN_POINT ( 'NONE',  ( 0.3999999999999568345, 2.500000000000000000, -3.537306695894649966 ) ) ;
#90406=AXIS2_PLACEMENT_3D ( 'NONE', #114455, #59437, #20133 ) ;
#90407=VERTEX_POINT ( 'NONE', #87034 ) ;
#90408=DIRECTION ( 'NONE',  ( 0.000000000000000000, 0.000000000000000000, 1.000000000000000000 ) ) ;
#90409=DIRECTION ( 'NONE',  ( -0.000000000000000000, -1.000000000000000000, -0.000000000000000000 ) ) ;
#90410=AXIS2_PLACEMENT_3D ( 'NONE', #6420, #54907, #13688 ) ;
#90411=VERTEX_POINT ( 'NONE', #26836 ) ;
#90412=DIRECTION ( 'NONE',  ( 0.000000000000000000, 0.000000000000000000, 1.000000000000000000 ) ) ;
#90413=DIRECTION ( 'NONE',  ( 0.000000000000000000, 0.000000000000000000, 1.000000000000000000 ) ) ;
#90414=DIRECTION ( 'NONE',  ( 0.000000000000000000, -0.000000000000000000, 1.000000000000000000 ) ) ;
#90415=DIRECTION ( 'NONE',  ( 0.000000000000000000, 0.000000000000000000, 1.000000000000000000 ) ) ;
#90416=DIRECTION ( 'NONE',  ( -0.000000000000000000, -1.000000000000000000, -0.000000000000000000 ) ) ;
#90417=ORIENTED_EDGE ( 'NONE', *, *, #17666, .T. ) ;
#90418=CIRCLE ( 'NONE', #40279, 0.09999999999999982514 ) ;
#90419=CARTESIAN_POINT ( 'NONE',  ( 65.40463321312788025, 3.824478825999977794, -5.306487653624172296 ) ) ;
#90420=DIRECTION ( 'NONE',  ( 0.000000000000000000, 0.000000000000000000, -1.000000000000000000 ) ) ;
#90421=LINE ( 'NONE', #48594, #36606 ) ;
#90422=LINE ( 'NONE', #60982, #16645 ) ;
#90423=EDGE_CURVE ( 'NONE', #53181, #19084, #77138, .T. ) ;
#90424=ORIENTED_EDGE ( 'NONE', *, *, #1396, .T. ) ;
#90425=AXIS2_PLACEMENT_3D ( 'NONE', #104663, #74577, #86311 ) ;
#90426=AXIS2_PLACEMENT_3D ( 'NONE', #383, #125635, #50164 ) ;
#90427=ORIENTED_EDGE ( 'NONE', *, *, #108413, .T. ) ;
#90428=DIRECTION ( 'NONE',  ( 0.000000000000000000, 0.000000000000000000, 1.000000000000000000 ) ) ;
#90429=LINE ( 'NONE', #40735, #63384 ) ;
#90430=FACE_OUTER_BOUND ( 'NONE', #79266, .T. ) ;
#90431=VERTEX_POINT ( 'NONE', #16342 ) ;
#90432=ADVANCED_FACE ( 'NONE', ( #45835 ), #6506, .T. ) ;
#90433=CONICAL_SURFACE ( 'NONE', #96698, 0.09999999999999999167, 0.003490658503988666988 ) ;
#90434=CARTESIAN_POINT ( 'NONE',  ( 6.649999999999931966, 2.500000000000000000, -5.702370205355749455 ) ) ;
#90435=CIRCLE ( 'NONE', #42347, 0.06509327318403745899 ) ;
#90436=AXIS2_PLACEMENT_3D ( 'NONE', #114239, #74960, #95890 ) ;
#90437=DIRECTION ( 'NONE',  ( 0.000000000000000000, 1.000000000000000000, 0.000000000000000000 ) ) ;
#90438=AXIS2_PLACEMENT_3D ( 'NONE', #26770, #115788, #116420 ) ;
#90439=ORIENTED_EDGE ( 'NONE', *, *, #61067, .F. ) ;
#90440=AXIS2_PLACEMENT_3D ( 'NONE', #90626, #40918, #28500 ) ;
#90441=ADVANCED_FACE ( 'NONE', ( #80460 ), #3971, .T. ) ;
#90442=AXIS2_PLACEMENT_3D ( 'NONE', #78145, #29049, #57860 ) ;
#90443=CARTESIAN_POINT ( 'NONE',  ( -12.09999999999999609, 2.500000000000000000, -5.022947341949751454 ) ) ;
#90444=ADVANCED_FACE ( 'NONE', ( #78537 ), #119084, .T. ) ;
#90445=ORIENTED_EDGE ( 'NONE', *, *, #64221, .T. ) ;
#90446=CONICAL_SURFACE ( 'NONE', #63278, 0.09999999999999982514, 0.003490658503988666988 ) ;
#90447=CARTESIAN_POINT ( 'NONE',  ( -5.000000000000022204, 2.500000000000000000, 3.537306695894645081 ) ) ;
#90449=CARTESIAN_POINT ( 'NONE',  ( 7.099999999999928590, 2.500000000000000000, -4.230127018922201998 ) ) ;
#90450=CARTESIAN_POINT ( 'NONE',  ( -0.2000000000000339284, 2.500000000000000000, -0.4464101615137759382 ) ) ;
#90451=ADVANCED_FACE ( 'NONE', ( #29419 ), #120377, .T. ) ;
#90452=EDGE_LOOP ( 'NONE', ( #93172, #102945, #92054, #84077 ) ) ;
#90453=ORIENTED_EDGE ( 'NONE', *, *, #7205, .F. ) ;
#90454=EDGE_CURVE ( 'NONE', #69316, #97467, #28780, .T. ) ;
#90455=FACE_OUTER_BOUND ( 'NONE', #36994, .T. ) ;
#90456=DIRECTION ( 'NONE',  ( 0.000000000000000000, 0.000000000000000000, 1.000000000000000000 ) ) ;
#90457=ORIENTED_EDGE ( 'NONE', *, *, #56214, .T. ) ;
#90459=CARTESIAN_POINT ( 'NONE',  ( -5.600000000000020073, 2.500000000000000000, -0.3464101615137782364 ) ) ;
#90460=DIRECTION ( 'NONE',  ( 0.000000000000000000, 0.000000000000000000, 1.000000000000000000 ) ) ;
#90461=LINE ( 'NONE', #91125, #49529 ) ;
#90463=CARTESIAN_POINT ( 'NONE',  ( 87.50000000000001421, 3.975350567648425759, 6.360562287258741065 ) ) ;
#90464=CARTESIAN_POINT ( 'NONE',  ( 4.999999999999935163, 12.50000000000000000, 3.702399969078682407 ) ) ;
#90465=DIRECTION ( 'NONE',  ( -0.000000000000000000, -1.000000000000000000, -0.000000000000000000 ) ) ;
#90466=CONICAL_SURFACE ( 'NONE', #77962, 0.1000000000000000472, 0.003490658503988666988 ) ;
#90467=CIRCLE ( 'NONE', #84215, 0.06509327318403745899 ) ;
#90468=AXIS2_PLACEMENT_3D ( 'NONE', #52487, #91135, #2092 ) ;
#90470=ORIENTED_EDGE ( 'NONE', *, *, #29176, .F. ) ;
#90471=VERTEX_POINT ( 'NONE', #60179 ) ;
#90472=CARTESIAN_POINT ( 'NONE',  ( -13.09999999999999254, 2.500000000000000000, -4.776537180435974861 ) ) ;
#90473=DIRECTION ( 'NONE',  ( 0.000000000000000000, -0.9999939076577903929, 0.003490651415223739937 ) ) ;
#90474=DIRECTION ( 'NONE',  ( -0.000000000000000000, 1.000000000000000000, -0.000000000000000000 ) ) ;
#90475=ORIENTED_EDGE ( 'NONE', *, *, #74835, .T. ) ;
#90476=ORIENTED_EDGE ( 'NONE', *, *, #68476, .T. ) ;
#90477=FACE_BOUND ( 'NONE', #44804, .T. ) ;
#90478=ORIENTED_EDGE ( 'NONE', *, *, #51772, .F. ) ;
#90479=AXIS2_PLACEMENT_3D ( 'NONE', #50375, #119119, #109953 ) ;
#90480=CARTESIAN_POINT ( 'NONE',  ( -0.8500000000000386136, 12.50000000000000000, 7.188010851410848723 ) ) ;
#90482=CIRCLE ( 'NONE', #29864, 0.06509327318403745899 ) ;
#90483=AXIS2_PLACEMENT_3D ( 'NONE', #19679, #30155, #89700 ) ;
#90484=FACE_OUTER_BOUND ( 'NONE', #98144, .T. ) ;
#90485=CARTESIAN_POINT ( 'NONE',  ( -3.100000000000028511, 2.500000000000000000, 0.3464101615137736845 ) ) ;
#90486=AXIS2_PLACEMENT_3D ( 'NONE', #58407, #110073, #18462 ) ;
#90487=CARTESIAN_POINT ( 'NONE',  ( -13.14999999999999147, 2.500000000000000000, 1.818653347947325472 ) ) ;
#90488=PLANE ( 'NONE',  #29764 ) ;
#90489=CARTESIAN_POINT ( 'NONE',  ( 0.3999999999999563904, 2.500000000000000000, 5.022947341949748790 ) ) ;
#90490=LINE ( 'NONE', #121257, #10167 ) ;
#90491=CARTESIAN_POINT ( 'NONE',  ( 9.999999999999948486, 2.500000000000000000, 4.330127018922196314 ) ) ;
#90492=VECTOR ( 'NONE', #118310, 1000.000000000000000 ) ;
#90493=LINE ( 'NONE', #42061, #84811 ) ;
#90494=ADVANCED_FACE ( 'NONE', ( #107324 ), #112651, .T. ) ;
#90495=AXIS2_PLACEMENT_3D ( 'NONE', #31193, #101849, #22018 ) ;
#90496=VERTEX_POINT ( 'NONE', #57595 ) ;
#90497=EDGE_LOOP ( 'NONE', ( #63858, #22556, #41885, #31004 ) ) ;
#90498=ORIENTED_EDGE ( 'NONE', *, *, #100237, .T. ) ;
#90499=AXIS2_PLACEMENT_3D ( 'NONE', #1191, #82995, #41143 ) ;
#90500=EDGE_LOOP ( 'NONE', ( #83941, #101371 ) ) ;
#90501=AXIS2_PLACEMENT_3D ( 'NONE', #36639, #116454, #28089 ) ;
#90502=CIRCLE ( 'NONE', #42507, 0.06509327318403745899 ) ;
#90503=CARTESIAN_POINT ( 'NONE',  ( 11.64999999999990266, 2.500000000000000000, -6.395190528383301931 ) ) ;
#90504=EDGE_CURVE ( 'NONE', #114462, #24394, #72937, .T. ) ;
#90505=CARTESIAN_POINT ( 'NONE',  ( -1.250000000000001554, 12.50000000000000000, 2.165063509461097713 ) ) ;
#90506=ADVANCED_FACE ( 'NONE', ( #117765 ), #128273, .T. ) ;
#90507=ORIENTED_EDGE ( 'NONE', *, *, #33434, .F. ) ;
#90509=EDGE_LOOP ( 'NONE', ( #113339, #1632, #61141, #90931 ) ) ;
#90510=CIRCLE ( 'NONE', #42512, 0.06509327318403745899 ) ;
#90511=EDGE_CURVE ( 'NONE', #38970, #100810, #26976, .T. ) ;
#90512=CARTESIAN_POINT ( 'NONE',  ( -0.6000000000000383915, 12.50000000000000000, -4.676537180435977881 ) ) ;
#90513=ADVANCED_FACE ( 'NONE', ( #68040 ), #54164, .T. ) ;
#90514=CARTESIAN_POINT ( 'NONE',  ( -2.300000000000033573, 12.50000000000000000, 4.676537180435972552 ) ) ;
#90515=CIRCLE ( 'NONE', #96761, 0.1000000000000002554 ) ;
#90516=DIRECTION ( 'NONE',  ( 0.000000000000000000, 0.000000000000000000, 1.000000000000000000 ) ) ;
#90517=DIRECTION ( 'NONE',  ( 0.000000000000000000, 0.000000000000000000, -1.000000000000000000 ) ) ;
#90518=EDGE_CURVE ( 'NONE', #55517, #116823, #18295, .T. ) ;
#90519=DIRECTION ( 'NONE',  ( -0.000000000000000000, 1.000000000000000000, -0.000000000000000000 ) ) ;
#90520=DIRECTION ( 'NONE',  ( -0.000000000000000000, 1.000000000000000000, -0.000000000000000000 ) ) ;
#90521=DIRECTION ( 'NONE',  ( 0.000000000000000000, 1.000000000000000000, 0.000000000000000000 ) ) ;
#90522=VERTEX_POINT ( 'NONE', #58244 ) ;
#90523=DIRECTION ( 'NONE',  ( 0.000000000000000000, 1.000000000000000000, 0.000000000000000000 ) ) ;
#90524=EDGE_CURVE ( 'NONE', #78169, #72699, #70887, .T. ) ;
#90525=VERTEX_POINT ( 'NONE', #89621 ) ;
#90526=ADVANCED_FACE ( 'NONE', ( #109248 ), #16480, .T. ) ;
#90527=VERTEX_POINT ( 'NONE', #9126 ) ;
#90528=EDGE_LOOP ( 'NONE', ( #16241, #52804 ) ) ;
#90530=AXIS2_PLACEMENT_3D ( 'NONE', #53672, #73302, #62221 ) ;
#90531=VERTEX_POINT ( 'NONE', #88978 ) ;
#90532=ORIENTED_EDGE ( 'NONE', *, *, #78530, .T. ) ;
#90533=DIRECTION ( 'NONE',  ( -4.274815082592931898E-19, -0.9999939076577903929, -0.003490651415223739937 ) ) ;
#90534=AXIS2_PLACEMENT_3D ( 'NONE', #22037, #41684, #121487 ) ;
#90535=DIRECTION ( 'NONE',  ( 0.000000000000000000, 0.000000000000000000, 1.000000000000000000 ) ) ;
#90536=FACE_OUTER_BOUND ( 'NONE', #106475, .T. ) ;
#90537=CIRCLE ( 'NONE', #38325, 0.09999999999999982514 ) ;
#90538=DIRECTION ( 'NONE',  ( 0.000000000000000000, -0.9999939076577903929, 0.003490651415223739937 ) ) ;
#90539=DIRECTION ( 'NONE',  ( 0.000000000000000000, 0.000000000000000000, -1.000000000000000000 ) ) ;
#90540=CIRCLE ( 'NONE', #98848, 0.06509327318403745899 ) ;
#90541=AXIS2_PLACEMENT_3D ( 'NONE', #36336, #105034, #16647 ) ;
#90542=DIRECTION ( 'NONE',  ( -4.274815082592931898E-19, -0.9999939076577903929, -0.003490651415223739937 ) ) ;
#90543=EDGE_CURVE ( 'NONE', #38720, #7794, #104240, .T. ) ;
#90544=CARTESIAN_POINT ( 'NONE',  ( -12.49999999999995914, 2.500000000000000000, -4.430127018922199511 ) ) ;
#90545=AXIS2_PLACEMENT_3D ( 'NONE', #56118, #14881, #67198 ) ;
#90546=ORIENTED_EDGE ( 'NONE', *, *, #22000, .F. ) ;
#90547=CARTESIAN_POINT ( 'NONE',  ( 21.24748443165277223, 0.7426079187842503648, 4.181982372968837680 ) ) ;
#90548=CIRCLE ( 'NONE', #67544, 0.09999999999999982514 ) ;
#90549=ORIENTED_EDGE ( 'NONE', *, *, #65318, .T. ) ;
#90551=CARTESIAN_POINT ( 'NONE',  ( 0.8499999999999550138, 2.500000000000000000, -5.802370205355749988 ) ) ;
#90552=AXIS2_PLACEMENT_3D ( 'NONE', #67969, #47709, #18223 ) ;
#90553=ORIENTED_EDGE ( 'NONE', *, *, #111671, .T. ) ;
#90554=AXIS2_PLACEMENT_3D ( 'NONE', #117910, #58375, #98270 ) ;
#90555=DIRECTION ( 'NONE',  ( 0.000000000000000000, 0.000000000000000000, 1.000000000000000000 ) ) ;
#90556=DIRECTION ( 'NONE',  ( 0.000000000000000000, -0.9999939076577903929, 0.003490651415223739937 ) ) ;
#90557=ORIENTED_EDGE ( 'NONE', *, *, #84359, .F. ) ;
#90558=AXIS2_PLACEMENT_3D ( 'NONE', #31815, #120197, #81554 ) ;
#90559=DIRECTION ( 'NONE',  ( -0.000000000000000000, 1.000000000000000000, -0.000000000000000000 ) ) ;
#90560=VERTEX_POINT ( 'NONE', #99455 ) ;
#90561=ORIENTED_EDGE ( 'NONE', *, *, #97697, .F. ) ;
#90562=DIRECTION ( 'NONE',  ( -0.000000000000000000, -1.000000000000000000, -0.000000000000000000 ) ) ;
#90563=DIRECTION ( 'NONE',  ( 0.000000000000000000, -0.000000000000000000, 1.000000000000000000 ) ) ;
#90564=LINE ( 'NONE', #900, #41820 ) ;
#90565=DIRECTION ( 'NONE',  ( 0.000000000000000000, -0.9999939076577903929, 0.003490651415223739937 ) ) ;
#90566=AXIS2_PLACEMENT_3D ( 'NONE', #84656, #82742, #112832 ) ;
#90567=DIRECTION ( 'NONE',  ( -0.000000000000000000, 1.000000000000000000, -0.000000000000000000 ) ) ;
#90568=EDGE_CURVE ( 'NONE', #97131, #65281, #9770, .T. ) ;
#90569=EDGE_LOOP ( 'NONE', ( #115120, #69079 ) ) ;
#90570=CARTESIAN_POINT ( 'NONE',  ( 3.949999999999942446, 12.50000000000000000, -2.446380397790840266 ) ) ;
#90571=VECTOR ( 'NONE', #12974, 1000.000000000000000 ) ;
#90573=CONICAL_SURFACE ( 'NONE', #42480, 0.1000000000000002554, 0.003490658503988666988 ) ;
#90574=DIRECTION ( 'NONE',  ( -0.000000000000000000, 1.000000000000000000, -0.000000000000000000 ) ) ;
#90575=DIRECTION ( 'NONE',  ( 0.000000000000000000, 1.000000000000000000, 0.000000000000000000 ) ) ;
#90579=CARTESIAN_POINT ( 'NONE',  ( 6.849999999999927702, 12.50000000000000000, 2.511473670974873507 ) ) ;
#90581=AXIS2_PLACEMENT_3D ( 'NONE', #4466, #44419, #41861 ) ;
#90582=DIRECTION ( 'NONE',  ( -0.000000000000000000, -1.000000000000000000, -0.000000000000000000 ) ) ;
#90583=VECTOR ( 'NONE', #12299, 1000.000000000000000 ) ;
#90584=VERTEX_POINT ( 'NONE', #50341 ) ;
#90585=CONICAL_SURFACE ( 'NONE', #59321, 0.1000000000000002554, 0.003490658503988666988 ) ;
#90586=DIRECTION ( 'NONE',  ( -0.000000000000000000, 1.000000000000000000, -0.000000000000000000 ) ) ;
#90587=DIRECTION ( 'NONE',  ( 0.000000000000000000, 0.000000000000000000, 1.000000000000000000 ) ) ;
#90588=DIRECTION ( 'NONE',  ( -0.000000000000000000, 1.000000000000000000, -0.000000000000000000 ) ) ;
#90589=CONICAL_SURFACE ( 'NONE', #709, 0.1000000000000000472, 0.003490658503988666988 ) ;
#90590=VERTEX_POINT ( 'NONE', #90242 ) ;
#90591=CARTESIAN_POINT ( 'NONE',  ( 11.24999999999990763, 12.50000000000000000, -7.188010851410854052 ) ) ;
#90592=ORIENTED_EDGE ( 'NONE', *, *, #119407, .F. ) ;
#90593=VECTOR ( 'NONE', #298, 1000.000000000000000 ) ;
#90594=AXIS2_PLACEMENT_3D ( 'NONE', #84102, #35037, #93939 ) ;
#90595=ORIENTED_EDGE ( 'NONE', *, *, #33871, .F. ) ;
#90596=CONICAL_SURFACE ( 'NONE', #82300, 0.1000000000000002554, 0.003490658503988666988 ) ;
#90597=CARTESIAN_POINT ( 'NONE',  ( 2.949999999999945111, 2.500000000000000000, 2.165063509461097713 ) ) ;
#90598=CONICAL_SURFACE ( 'NONE', #76037, 0.1000000000000002554, 0.003490658503988666988 ) ;
#90599=ORIENTED_EDGE ( 'NONE', *, *, #48595, .F. ) ;
#90600=FACE_OUTER_BOUND ( 'NONE', #6812, .T. ) ;
#90601=DIRECTION ( 'NONE',  ( -0.000000000000000000, 1.000000000000000000, -0.000000000000000000 ) ) ;
#90602=EDGE_LOOP ( 'NONE', ( #95373, #110955 ) ) ;
#90603=ADVANCED_FACE ( 'NONE', ( #580 ), #123114, .T. ) ;
#90604=FACE_OUTER_BOUND ( 'NONE', #8093, .T. ) ;
#90605=DIRECTION ( 'NONE',  ( 0.000000000000000000, 1.000000000000000000, 0.000000000000000000 ) ) ;
#90606=CARTESIAN_POINT ( 'NONE',  ( 4.349999999999939249, 12.50000000000000000, 2.511473670974873507 ) ) ;
#90607=EDGE_CURVE ( 'NONE', #89818, #73855, #100134, .T. ) ;
#90608=EDGE_CURVE ( 'NONE', #103695, #103569, #71259, .T. ) ;
#90609=ORIENTED_EDGE ( 'NONE', *, *, #91360, .F. ) ;
#90610=ORIENTED_EDGE ( 'NONE', *, *, #126161, .T. ) ;
#90611=ORIENTED_EDGE ( 'NONE', *, *, #122700, .T. ) ;
#90612=DIRECTION ( 'NONE',  ( 0.000000000000000000, 0.000000000000000000, 1.000000000000000000 ) ) ;
#90613=CARTESIAN_POINT ( 'NONE',  ( -9.999999999999971578, 12.50000000000000000, -4.330127018922197202 ) ) ;
#90614=EDGE_CURVE ( 'NONE', #45894, #37222, #121012, .T. ) ;
#90615=EDGE_CURVE ( 'NONE', #104775, #97182, #12284, .T. ) ;
#90616=DIRECTION ( 'NONE',  ( 0.000000000000000000, 0.000000000000000000, 1.000000000000000000 ) ) ;
#90617=AXIS2_PLACEMENT_3D ( 'NONE', #127389, #128707, #16755 ) ;
#90618=ADVANCED_FACE ( 'NONE', ( #22190 ), #118903, .T. ) ;
#90619=FACE_BOUND ( 'NONE', #37380, .T. ) ;
#90620=EDGE_LOOP ( 'NONE', ( #30537, #69002 ) ) ;
#90621=EDGE_CURVE ( 'NONE', #51095, #18351, #102190, .T. ) ;
#90622=EDGE_CURVE ( 'NONE', #121481, #36772, #87684, .T. ) ;
#90623=CARTESIAN_POINT ( 'NONE',  ( -14.79999999999998472, 2.500000000000000000, 0.3464101615137758494 ) ) ;
#90624=DIRECTION ( 'NONE',  ( -4.274815082592931898E-19, -0.9999939076577903929, -0.003490651415223739937 ) ) ;
#90626=CARTESIAN_POINT ( 'NONE',  ( -7.500000000000011546, 2.500000000000000000, 3.637306695894644726 ) ) ;
#90627=AXIS2_PLACEMENT_3D ( 'NONE', #45385, #62450, #114744 ) ;
#90628=CARTESIAN_POINT ( 'NONE',  ( 0.3999999999999563904, 12.50000000000000000, 5.022947341949748790 ) ) ;
#90629=VECTOR ( 'NONE', #15527, 1000.000000000000000 ) ;
#90630=CIRCLE ( 'NONE', #65489, 0.1000000000000000056 ) ;
#90631=CONICAL_SURFACE ( 'NONE', #27943, 0.1000000000000000472, 0.003490658503988666988 ) ;
#90632=LINE ( 'NONE', #49444, #554 ) ;
#90633=DIRECTION ( 'NONE',  ( 0.000000000000000000, 0.000000000000000000, -1.000000000000000000 ) ) ;
#90634=DIRECTION ( 'NONE',  ( 0.000000000000000000, 0.000000000000000000, 1.000000000000000000 ) ) ;
#90635=EDGE_CURVE ( 'NONE', #13143, #108629, #98059, .T. ) ;
#90636=CARTESIAN_POINT ( 'NONE',  ( -2.900000000000029221, 2.500000000000000000, -4.922947341949753586 ) ) ;
#90637=DIRECTION ( 'NONE',  ( 0.000000000000000000, 0.000000000000000000, -1.000000000000000000 ) ) ;
#90638=AXIS2_PLACEMENT_3D ( 'NONE', #76586, #104112, #123726 ) ;
#90639=AXIS2_PLACEMENT_3D ( 'NONE', #104207, #83297, #53820 ) ;
#90640=AXIS2_PLACEMENT_3D ( 'NONE', #17189, #106251, #76798 ) ;
#90641=ORIENTED_EDGE ( 'NONE', *, *, #83216, .T. ) ;
#90642=EDGE_LOOP ( 'NONE', ( #44620, #93724 ) ) ;
#90643=VERTEX_POINT ( 'NONE', #20884 ) ;
#90644=EDGE_LOOP ( 'NONE', ( #129265, #114698, #54730, #28824 ) ) ;
#90645=CARTESIAN_POINT ( 'NONE',  ( 5.849999999999933920, 2.500000000000000000, -2.757883832488654097 ) ) ;
#90646=VECTOR ( 'NONE', #8437, 1000.000000000000000 ) ;
#90647=DIRECTION ( 'NONE',  ( -4.274815082592931898E-19, -0.9999939076577903929, -0.003490651415223739937 ) ) ;
#90648=ORIENTED_EDGE ( 'NONE', *, *, #67334, .F. ) ;
#90649=FACE_BOUND ( 'NONE', #89361, .T. ) ;
#90650=DIRECTION ( 'NONE',  ( -0.000000000000000000, -1.000000000000000000, -0.000000000000000000 ) ) ;
#90651=DIRECTION ( 'NONE',  ( 0.000000000000000000, 0.000000000000000000, 1.000000000000000000 ) ) ;
#90652=DIRECTION ( 'NONE',  ( -0.000000000000000000, 1.000000000000000000, -0.000000000000000000 ) ) ;
#90653=DIRECTION ( 'NONE',  ( 0.000000000000000000, 1.000000000000000000, 0.000000000000000000 ) ) ;
#90654=CARTESIAN_POINT ( 'NONE',  ( 5.199999999999933564, 12.50000000000000000, 3.983716857408420076 ) ) ;
#90655=DIRECTION ( 'NONE',  ( 0.000000000000000000, -0.9999939076577903929, 0.003490651415223739937 ) ) ;
#90656=LINE ( 'NONE', #21938, #78450 ) ;
#90657=DIRECTION ( 'NONE',  ( 0.000000000000000000, 1.000000000000000000, 0.000000000000000000 ) ) ;
#90658=ORIENTED_EDGE ( 'NONE', *, *, #105541, .F. ) ;
#90659=CONICAL_SURFACE ( 'NONE', #126165, 0.1000000000000000056, 0.003490658503988666988 ) ;
#90660=VERTEX_POINT ( 'NONE', #82396 ) ;
#90661=ORIENTED_EDGE ( 'NONE', *, *, #95505, .F. ) ;
#90662=ORIENTED_EDGE ( 'NONE', *, *, #46921, .T. ) ;
#90664=ORIENTED_EDGE ( 'NONE', *, *, #35213, .F. ) ;
#90665=FACE_OUTER_BOUND ( 'NONE', #84186, .T. ) ;
#90666=ADVANCED_FACE ( 'NONE', ( #1239 ), #92855, .T. ) ;
#90667=ORIENTED_EDGE ( 'NONE', *, *, #63505, .F. ) ;
#90668=CIRCLE ( 'NONE', #34256, 0.06509327318403745899 ) ;
#90670=CIRCLE ( 'NONE', #4972, 0.1000000000000002554 ) ;
#90671=AXIS2_PLACEMENT_3D ( 'NONE', #127332, #89333, #127960 ) ;
#90672=EDGE_CURVE ( 'NONE', #113210, #112816, #112491, .T. ) ;
#90673=DIRECTION ( 'NONE',  ( 0.000000000000000000, 1.000000000000000000, 0.000000000000000000 ) ) ;
#90675=CARTESIAN_POINT ( 'NONE',  ( -9.800000000000006040, 2.500000000000000000, 0.4464101615137735513 ) ) ;
#90676=DIRECTION ( 'NONE',  ( 0.000000000000000000, 0.000000000000000000, 1.000000000000000000 ) ) ;
#90677=ADVANCED_FACE ( 'NONE', ( #12338 ), #96015, .T. ) ;
#90678=AXIS2_PLACEMENT_3D ( 'NONE', #93372, #111048, #22713 ) ;
#90679=ORIENTED_EDGE ( 'NONE', *, *, #38543, .F. ) ;
#90680=FACE_OUTER_BOUND ( 'NONE', #69828, .T. ) ;
#90681=CIRCLE ( 'NONE', #107402, 0.06509327318403745899 ) ;
#90682=ADVANCED_FACE ( 'NONE', ( #83671 ), #52922, .T. ) ;
#90683=ADVANCED_FACE ( 'NONE', ( #3182 ), #1913, .T. ) ;
#90685=VECTOR ( 'NONE', #103146, 1000.000000000000000 ) ;
#90686=ADVANCED_FACE ( 'NONE', ( #91555 ), #33297, .T. ) ;
#90687=ORIENTED_EDGE ( 'NONE', *, *, #90831, .F. ) ;
#90688=PLANE ( 'NONE',  #25989 ) ;
#90689=DIRECTION ( 'NONE',  ( 0.000000000000000000, 0.000000000000000000, 1.000000000000000000 ) ) ;
#90690=CARTESIAN_POINT ( 'NONE',  ( 4.149999999999936406, 2.500000000000000000, 6.395190528383296602 ) ) ;
#90691=CONICAL_SURFACE ( 'NONE', #44734, 0.1000000000000000472, 0.003490658503988666988 ) ;
#90692=ORIENTED_EDGE ( 'NONE', *, *, #98332, .F. ) ;
#90693=EDGE_CURVE ( 'NONE', #87945, #78195, #123215, .T. ) ;
#90694=ORIENTED_EDGE ( 'NONE', *, *, #89684, .F. ) ;
#90695=PLANE ( 'NONE',  #6650 ) ;
#90696=CARTESIAN_POINT ( 'NONE',  ( 1.249999999999952038, 12.50000000000000000, 5.802370205355744659 ) ) ;
#90697=CIRCLE ( 'NONE', #69767, 0.06509327318403745899 ) ;
#90698=LINE ( 'NONE', #69768, #85415 ) ;
#90699=AXIS2_PLACEMENT_3D ( 'NONE', #73266, #82463, #63454 ) ;
#90700=AXIS2_PLACEMENT_3D ( 'NONE', #127184, #48612, #29605 ) ;
#90701=LINE ( 'NONE', #51440, #90072 ) ;
#90702=VERTEX_POINT ( 'NONE', #76427 ) ;
#90703=DIRECTION ( 'NONE',  ( 0.000000000000000000, 0.000000000000000000, 1.000000000000000000 ) ) ;
#90704=VECTOR ( 'NONE', #14003, 1000.000000000000000 ) ;
#90705=ORIENTED_EDGE ( 'NONE', *, *, #128813, .T. ) ;
#90706=AXIS2_PLACEMENT_3D ( 'NONE', #59089, #38155, #86597 ) ;
#90707=CARTESIAN_POINT ( 'NONE',  ( 13.12246079422085288, -2.500000000000001332, 7.156134183588244824 ) ) ;
#90708=ORIENTED_EDGE ( 'NONE', *, *, #65098, .T. ) ;
#90709=CARTESIAN_POINT ( 'NONE',  ( 87.50000000000001421, 4.424430252271040587, 6.079088403633666537 ) ) ;
#90710=CARTESIAN_POINT ( 'NONE',  ( 0.3999999999999619971, 2.500000000000000000, -1.084202172485504434E-16 ) ) ;
#90711=DIRECTION ( 'NONE',  ( -0.000000000000000000, -1.000000000000000000, -0.000000000000000000 ) ) ;
#90712=ADVANCED_FACE ( 'NONE', ( #105234 ), #127411, .T. ) ;
#90713=CARTESIAN_POINT ( 'NONE',  ( 1.899999999999949507, 2.500000000000000000, 3.883716857408421319 ) ) ;
#90714=ORIENTED_EDGE ( 'NONE', *, *, #16495, .T. ) ;
#90715=DIRECTION ( 'NONE',  ( -0.000000000000000000, -1.000000000000000000, -0.000000000000000000 ) ) ;
#90716=CARTESIAN_POINT ( 'NONE',  ( 4.999999999999933387, 2.500000000000000000, 4.922947341949748257 ) ) ;
#90717=ORIENTED_EDGE ( 'NONE', *, *, #41866, .F. ) ;
#90718=VERTEX_POINT ( 'NONE', #115689 ) ;
#90719=AXIS2_PLACEMENT_3D ( 'NONE', #110503, #100667, #10997 ) ;
#90720=CIRCLE ( 'NONE', #105298, 0.1000000000000000472 ) ;
#90721=VERTEX_POINT ( 'NONE', #116332 ) ;
#90722=DIRECTION ( 'NONE',  ( 0.000000000000000000, -0.9999939076577903929, 0.003490651415223739937 ) ) ;
#90723=DIRECTION ( 'NONE',  ( 0.000000000000000000, 0.000000000000000000, 1.000000000000000000 ) ) ;
#90724=DIRECTION ( 'NONE',  ( -0.000000000000000000, 1.000000000000000000, -0.000000000000000000 ) ) ;
#90726=FACE_OUTER_BOUND ( 'NONE', #69756, .T. ) ;
#90727=DIRECTION ( 'NONE',  ( -0.000000000000000000, 1.000000000000000000, -0.000000000000000000 ) ) ;
#90728=AXIS2_PLACEMENT_3D ( 'NONE', #94454, #95123, #15238 ) ;
#90729=AXIS2_PLACEMENT_3D ( 'NONE', #102484, #92663, #122772 ) ;
#90730=CARTESIAN_POINT ( 'NONE',  ( 6.649999999999930189, 12.50000000000000000, -2.857883832488653741 ) ) ;
#90731=ADVANCED_FACE ( 'NONE', ( #15551 ), #39608, .T. ) ;
#90732=AXIS2_PLACEMENT_3D ( 'NONE', #70519, #31262, #110443 ) ;
#90733=DIRECTION ( 'NONE',  ( 0.000000000000000000, 0.000000000000000000, -1.000000000000000000 ) ) ;
#90734=DIRECTION ( 'NONE',  ( 0.000000000000000000, 0.000000000000000000, 1.000000000000000000 ) ) ;
#90735=CIRCLE ( 'NONE', #51038, 0.1000000000000002554 ) ;
#90736=CIRCLE ( 'NONE', #99062, 0.1000000000000002554 ) ;
#90737=ORIENTED_EDGE ( 'NONE', *, *, #40319, .F. ) ;
#90738=DIRECTION ( 'NONE',  ( 0.000000000000000000, -0.000000000000000000, 1.000000000000000000 ) ) ;
#90739=EDGE_CURVE ( 'NONE', #105289, #126127, #46974, .T. ) ;
#90740=CARTESIAN_POINT ( 'NONE',  ( -4.119968255444916849E-14, 12.50000000000000000, 3.637306695894644726 ) ) ;
#90741=LINE ( 'NONE', #1065, #90279 ) ;
#90742=DIRECTION ( 'NONE',  ( 0.000000000000000000, -0.000000000000000000, 1.000000000000000000 ) ) ;
#90743=ORIENTED_EDGE ( 'NONE', *, *, #123945, .F. ) ;
#90744=PLANE ( 'NONE',  #46637 ) ;
#90745=DIRECTION ( 'NONE',  ( 0.000000000000000000, 0.000000000000000000, -1.000000000000000000 ) ) ;
#90746=DIRECTION ( 'NONE',  ( -4.274815082592931898E-19, -0.9999939076577903929, -0.003490651415223739937 ) ) ;
#90747=ORIENTED_EDGE ( 'NONE', *, *, #95975, .T. ) ;
#90748=AXIS2_PLACEMENT_3D ( 'NONE', #91175, #52540, #91820 ) ;
#90749=VECTOR ( 'NONE', #36491, 1000.000000000000000 ) ;
#90750=VERTEX_POINT ( 'NONE', #45683 ) ;
#90751=CARTESIAN_POINT ( 'NONE',  ( 8.149999999999920419, 2.500000000000000000, 6.048780366869521252 ) ) ;
#90753=ORIENTED_EDGE ( 'NONE', *, *, #60921, .F. ) ;
#90754=CARTESIAN_POINT ( 'NONE',  ( 10.19999999999991047, 2.500000000000000000, -3.983716857408426293 ) ) ;
#90755=CARTESIAN_POINT ( 'NONE',  ( -14.34999999999998543, 12.50000000000000000, 2.511473670974877503 ) ) ;
#90756=FACE_OUTER_BOUND ( 'NONE', #108805, .T. ) ;
#90757=CIRCLE ( 'NONE', #36402, 0.1000000000000000472 ) ;
#90758=CARTESIAN_POINT ( 'NONE',  ( 10.84999999999990905, 2.500000000000000000, 1.472243186433545459 ) ) ;
#90759=CONICAL_SURFACE ( 'NONE', #76101, 0.09999999999999982514, 0.003490658503988666988 ) ;
#90760=EDGE_LOOP ( 'NONE', ( #52319, #34615 ) ) ;
#90761=ADVANCED_FACE ( 'NONE', ( #113777 ), #104419, .T. ) ;
#90762=FACE_OUTER_BOUND ( 'NONE', #121055, .T. ) ;
#90763=ORIENTED_EDGE ( 'NONE', *, *, #60221, .F. ) ;
#90764=LINE ( 'NONE', #1093, #115410 ) ;
#90765=DIRECTION ( 'NONE',  ( -4.274815082592931898E-19, -0.9999939076577903929, -0.003490651415223739937 ) ) ;
#90766=EDGE_CURVE ( 'NONE', #113146, #20664, #4424, .T. ) ;
#90767=VERTEX_POINT ( 'NONE', #95422 ) ;
#90768=CIRCLE ( 'NONE', #34362, 0.1000000000000002554 ) ;
#90769=ORIENTED_EDGE ( 'NONE', *, *, #64312, .F. ) ;
#90770=ORIENTED_EDGE ( 'NONE', *, *, #83409, .T. ) ;
#90771=ORIENTED_EDGE ( 'NONE', *, *, #53531, .F. ) ;
#90772=CARTESIAN_POINT ( 'NONE',  ( 10.39999999999991331, 12.50000000000000000, 0.06509327318403504425 ) ) ;
#90773=CARTESIAN_POINT ( 'NONE',  ( -5.450000000000023270, 12.50000000000000000, -6.430097255199264339 ) ) ;
#90774=ADVANCED_FACE ( 'NONE', ( #24750 ), #84305, .T. ) ;
#90775=EDGE_CURVE ( 'NONE', #18351, #51095, #31279, .T. ) ;
#90776=DIRECTION ( 'NONE',  ( 0.000000000000000000, 0.000000000000000000, -1.000000000000000000 ) ) ;
#90777=ADVANCED_FACE ( 'NONE', ( #35855 ), #112751, .T. ) ;
#90778=FACE_BOUND ( 'NONE', #90958, .T. ) ;
#90779=EDGE_CURVE ( 'NONE', #47037, #113203, #114779, .T. ) ;
#90780=DIRECTION ( 'NONE',  ( -0.000000000000000000, 1.000000000000000000, -0.000000000000000000 ) ) ;
#90782=DIRECTION ( 'NONE',  ( -0.000000000000000000, 1.000000000000000000, -0.000000000000000000 ) ) ;
#90783=DIRECTION ( 'NONE',  ( -0.000000000000000000, -1.000000000000000000, -0.000000000000000000 ) ) ;
#90785=AXIS2_PLACEMENT_3D ( 'NONE', #59742, #79996, #97061 ) ;
#90786=DIRECTION ( 'NONE',  ( 0.000000000000000000, 0.000000000000000000, -1.000000000000000000 ) ) ;
#90787=CARTESIAN_POINT ( 'NONE',  ( -4.150000000000025224, 2.500000000000000000, 7.088010851410848190 ) ) ;
#90788=AXIS2_PLACEMENT_3D ( 'NONE', #34819, #45912, #125728 ) ;
#90789=EDGE_CURVE ( 'NONE', #119719, #6241, #96683, .T. ) ;
#90790=CARTESIAN_POINT ( 'NONE',  ( -12.09999999999999609, 12.50000000000000000, 1.734723475976807094E-15 ) ) ;
#90791=AXIS2_PLACEMENT_3D ( 'NONE', #54706, #4964, #44916 ) ;
#90792=EDGE_CURVE ( 'NONE', #5713, #7097, #118993, .T. ) ;
#90793=EDGE_CURVE ( 'NONE', #79722, #113934, #34588, .T. ) ;
#90794=DIRECTION ( 'NONE',  ( 0.000000000000000000, -0.000000000000000000, 1.000000000000000000 ) ) ;
#90795=VERTEX_POINT ( 'NONE', #6358 ) ;
#90796=ORIENTED_EDGE ( 'NONE', *, *, #33947, .T. ) ;
#90797=VERTEX_POINT ( 'NONE', #73845 ) ;
#90798=ORIENTED_EDGE ( 'NONE', *, *, #2323, .T. ) ;
#90799=ORIENTED_EDGE ( 'NONE', *, *, #90143, .T. ) ;
#90800=DIRECTION ( 'NONE',  ( 0.000000000000000000, 0.000000000000000000, 1.000000000000000000 ) ) ;
#90801=CARTESIAN_POINT ( 'NONE',  ( -10.45000000000000107, 12.50000000000000000, 6.495190528383297135 ) ) ;
#90802=EDGE_LOOP ( 'NONE', ( #124537, #18208, #24334, #116472 ) ) ;
#90803=FACE_BOUND ( 'NONE', #113530, .T. ) ;
#90804=CARTESIAN_POINT ( 'NONE',  ( -3.550000000000028244, 2.500000000000000000, 2.511473670974873507 ) ) ;
#90805=CIRCLE ( 'NONE', #34398, 0.06509327318403745899 ) ;
#90806=CIRCLE ( 'NONE', #3081, 0.09999999999999982514 ) ;
#90807=CIRCLE ( 'NONE', #65665, 0.06509327318403745899 ) ;
#90808=ORIENTED_EDGE ( 'NONE', *, *, #13371, .T. ) ;
#90809=CARTESIAN_POINT ( 'NONE',  ( -8.350000000000012079, 12.50000000000000000, -2.792790559304616504 ) ) ;
#90810=LINE ( 'NONE', #71824, #103750 ) ;
#90811=CARTESIAN_POINT ( 'NONE',  ( 9.199999999999919353, 2.500000000000000000, 0.09999999999999772959 ) ) ;
#90812=CARTESIAN_POINT ( 'NONE',  ( -11.84999999999999787, 12.50000000000000000, -1.883746621131359378 ) ) ;
#90813=ORIENTED_EDGE ( 'NONE', *, *, #6966, .T. ) ;
#90814=DIRECTION ( 'NONE',  ( 0.000000000000000000, 0.000000000000000000, -1.000000000000000000 ) ) ;
#90815=CONICAL_SURFACE ( 'NONE', #53179, 0.1000000000000002554, 0.003490658503988666988 ) ;
#90816=AXIS2_PLACEMENT_3D ( 'NONE', #50298, #108568, #9727 ) ;
#90817=VECTOR ( 'NONE', #34386, 1000.000000000000000 ) ;
#90819=ORIENTED_EDGE ( 'NONE', *, *, #42020, .F. ) ;
#90820=FACE_OUTER_BOUND ( 'NONE', #101367, .T. ) ;
#90821=PLANE ( 'NONE',  #47731 ) ;
#90822=VERTEX_POINT ( 'NONE', #56124 ) ;
#90823=CARTESIAN_POINT ( 'NONE',  ( 11.24999999999990763, 2.500000000000000000, -7.188010851410854052 ) ) ;
#90824=CIRCLE ( 'NONE', #61600, 0.09999999999999982514 ) ;
#90825=CARTESIAN_POINT ( 'NONE',  ( -7.300000000000018474, 12.50000000000000000, 0.3464101615137735735 ) ) ;
#90826=FACE_OUTER_BOUND ( 'NONE', #83946, .T. ) ;
#90827=CARTESIAN_POINT ( 'NONE',  ( 1.649999999999949729, 12.50000000000000000, 7.188010851410848723 ) ) ;
#90828=CIRCLE ( 'NONE', #34420, 0.06509327318403745899 ) ;
#90829=ORIENTED_EDGE ( 'NONE', *, *, #116484, .F. ) ;
#90830=DIRECTION ( 'NONE',  ( -0.000000000000000000, -1.000000000000000000, -0.000000000000000000 ) ) ;
#90831=EDGE_CURVE ( 'NONE', #36682, #1853, #108529, .T. ) ;
#90832=EDGE_LOOP ( 'NONE', ( #65197, #104397, #4344, #2316 ) ) ;
#90833=DIRECTION ( 'NONE',  ( 0.000000000000000000, -0.000000000000000000, 1.000000000000000000 ) ) ;
#90834=EDGE_CURVE ( 'NONE', #21997, #25459, #52109, .T. ) ;
#90835=ORIENTED_EDGE ( 'NONE', *, *, #127160, .T. ) ;
#90836=CARTESIAN_POINT ( 'NONE',  ( 10.44999999999991402, 12.50000000000000000, -2.165063509461101710 ) ) ;
#90837=EDGE_CURVE ( 'NONE', #39963, #73967, #75087, .T. ) ;
#90838=VERTEX_POINT ( 'NONE', #54832 ) ;
#90839=CARTESIAN_POINT ( 'NONE',  ( -8.350000000000013856, 2.500000000000000000, -2.265063509461101798 ) ) ;
#90840=DIRECTION ( 'NONE',  ( 0.000000000000000000, 0.000000000000000000, -1.000000000000000000 ) ) ;
#90841=CARTESIAN_POINT ( 'NONE',  ( -10.85000000000000142, 12.50000000000000000, 2.165063509461097713 ) ) ;
#90842=DIRECTION ( 'NONE',  ( 0.000000000000000000, 1.000000000000000000, 0.000000000000000000 ) ) ;
#90843=DIRECTION ( 'NONE',  ( -0.000000000000000000, 1.000000000000000000, -0.000000000000000000 ) ) ;
#90844=CIRCLE ( 'NONE', #55340, 0.1000000000000000056 ) ;
#90845=VERTEX_POINT ( 'NONE', #96056 ) ;
#90846=EDGE_CURVE ( 'NONE', #83004, #76936, #129491, .T. ) ;
#90847=ORIENTED_EDGE ( 'NONE', *, *, #56479, .F. ) ;
#90848=ORIENTED_EDGE ( 'NONE', *, *, #72536, .T. ) ;
#90850=DIRECTION ( 'NONE',  ( 0.000000000000000000, 1.000000000000000000, 0.000000000000000000 ) ) ;
#90851=CARTESIAN_POINT ( 'NONE',  ( -8.550000000000013145, 2.500000000000000000, -1.818653347947326138 ) ) ;
#90852=ORIENTED_EDGE ( 'NONE', *, *, #26067, .F. ) ;
#90853=ORIENTED_EDGE ( 'NONE', *, *, #75879, .T. ) ;
#90854=VERTEX_POINT ( 'NONE', #12021 ) ;
#90855=CARTESIAN_POINT ( 'NONE',  ( 5.449999999999936229, 2.500000000000000000, -2.165063509461101710 ) ) ;
#90856=CIRCLE ( 'NONE', #59500, 0.1000000000000002554 ) ;
#90857=ORIENTED_EDGE ( 'NONE', *, *, #9592, .F. ) ;
#90858=CARTESIAN_POINT ( 'NONE',  ( 13.54999999999989768, 2.500000000000000000, -2.511473670974877948 ) ) ;
#90859=CARTESIAN_POINT ( 'NONE',  ( 5.199999999999935341, 2.500000000000000000, -3.883716857408426648 ) ) ;
#90860=FACE_OUTER_BOUND ( 'NONE', #23288, .T. ) ;
#90861=DIRECTION ( 'NONE',  ( 0.000000000000000000, 0.000000000000000000, -1.000000000000000000 ) ) ;
#90862=FACE_OUTER_BOUND ( 'NONE', #4374, .T. ) ;
#90863=CARTESIAN_POINT ( 'NONE',  ( 9.999999999999912959, 12.50000000000000000, 3.702399969078682407 ) ) ;
#90864=CARTESIAN_POINT ( 'NONE',  ( -2.300000000000033129, 2.500000000000000000, 3.883716857408420431 ) ) ;
#90865=EDGE_CURVE ( 'NONE', #129208, #81079, #69661, .T. ) ;
#90866=DIRECTION ( 'NONE',  ( 0.000000000000000000, 1.000000000000000000, 0.000000000000000000 ) ) ;
#90867=VERTEX_POINT ( 'NONE', #70315 ) ;
#90868=CIRCLE ( 'NONE', #59600, 0.09999999999999999167 ) ;
#90869=DIRECTION ( 'NONE',  ( 0.000000000000000000, -0.000000000000000000, 1.000000000000000000 ) ) ;
#90870=CARTESIAN_POINT ( 'NONE',  ( 5.199999999999933564, 12.50000000000000000, 0.3464101615137735735 ) ) ;
#90871=AXIS2_PLACEMENT_3D ( 'NONE', #34801, #114618, #96257 ) ;
#90872=ORIENTED_EDGE ( 'NONE', *, *, #73394, .T. ) ;
#90873=VERTEX_POINT ( 'NONE', #110234 ) ;
#90875=DIRECTION ( 'NONE',  ( -0.000000000000000000, 1.000000000000000000, -0.000000000000000000 ) ) ;
#90876=FACE_OUTER_BOUND ( 'NONE', #14477, .T. ) ;
#90878=CARTESIAN_POINT ( 'NONE',  ( -10.45000000000000462, 12.50000000000000000, -2.165063509461097713 ) ) ;
#90879=CONICAL_SURFACE ( 'NONE', #86669, 0.1000000000000000472, 0.003490658503988666988 ) ;
#90881=AXIS2_PLACEMENT_3D ( 'NONE', #85499, #86117, #55397 ) ;
#90882=EDGE_CURVE ( 'NONE', #5168, #116825, #12382, .T. ) ;
#90883=FACE_OUTER_BOUND ( 'NONE', #63308, .T. ) ;
#90884=CARTESIAN_POINT ( 'NONE',  ( 0.6499999999999561684, 12.50000000000000000, 2.576566944158910744 ) ) ;
#90885=AXIS2_PLACEMENT_3D ( 'NONE', #7243, #107396, #46532 ) ;
#90886=AXIS2_PLACEMENT_3D ( 'NONE', #31714, #21236, #42851 ) ;
#90887=PLANE ( 'NONE',  #29133 ) ;
#90888=VERTEX_POINT ( 'NONE', #40213 ) ;
#90889=EDGE_LOOP ( 'NONE', ( #115544, #87280, #50641, #66089 ) ) ;
#90890=EDGE_LOOP ( 'NONE', ( #2343, #101617, #86371, #91290 ) ) ;
#90891=ORIENTED_EDGE ( 'NONE', *, *, #53050, .T. ) ;
#90892=EDGE_CURVE ( 'NONE', #11640, #87436, #14520, .T. ) ;
#90893=ORIENTED_EDGE ( 'NONE', *, *, #112042, .T. ) ;
#90894=CARTESIAN_POINT ( 'NONE',  ( 10.84999999999990905, 12.50000000000000000, 2.857883832488649301 ) ) ;
#90895=CARTESIAN_POINT ( 'NONE',  ( -4.150000000000028777, 2.500000000000000000, -5.802370205355749988 ) ) ;
#90896=ORIENTED_EDGE ( 'NONE', *, *, #45744, .F. ) ;
#90897=PLANE ( 'NONE',  #75778 ) ;
#90899=CONICAL_SURFACE ( 'NONE', #74179, 0.09999999999999982514, 0.003490658503988666988 ) ;
#90900=AXIS2_PLACEMENT_3D ( 'NONE', #81553, #113593, #122766 ) ;
#90901=FACE_OUTER_BOUND ( 'NONE', #7182, .T. ) ;
#90902=DIRECTION ( 'NONE',  ( 0.000000000000000000, 0.000000000000000000, 1.000000000000000000 ) ) ;
#90903=ORIENTED_EDGE ( 'NONE', *, *, #90046, .T. ) ;
#90904=AXIS2_PLACEMENT_3D ( 'NONE', #27759, #118725, #18594 ) ;
#90905=AXIS2_PLACEMENT_3D ( 'NONE', #96603, #67133, #56677 ) ;
#90906=ADVANCED_FACE ( 'NONE', ( #50055 ), #125256, .T. ) ;
#90907=DIRECTION ( 'NONE',  ( 0.000000000000000000, 0.000000000000000000, 1.000000000000000000 ) ) ;
#90908=DIRECTION ( 'NONE',  ( 0.000000000000000000, 1.000000000000000000, 0.000000000000000000 ) ) ;
#90909=ORIENTED_EDGE ( 'NONE', *, *, #109264, .F. ) ;
#90910=AXIS2_PLACEMENT_3D ( 'NONE', #62390, #102313, #52554 ) ;
#90911=AXIS2_PLACEMENT_3D ( 'NONE', #66033, #16897, #85024 ) ;
#90912=AXIS2_PLACEMENT_3D ( 'NONE', #95222, #5530, #46114 ) ;
#90913=ORIENTED_EDGE ( 'NONE', *, *, #34644, .T. ) ;
#90914=ORIENTED_EDGE ( 'NONE', *, *, #27112, .T. ) ;
#90915=ORIENTED_EDGE ( 'NONE', *, *, #83752, .F. ) ;
#90916=DIRECTION ( 'NONE',  ( -0.000000000000000000, -1.000000000000000000, -0.000000000000000000 ) ) ;
#90917=CIRCLE ( 'NONE', #5225, 0.06509327318403745899 ) ;
#90918=DIRECTION ( 'NONE',  ( 0.000000000000000000, -0.9999939076577903929, 0.003490651415223739937 ) ) ;
#90919=DIRECTION ( 'NONE',  ( 0.000000000000000000, 0.000000000000000000, -1.000000000000000000 ) ) ;
#90920=AXIS2_PLACEMENT_3D ( 'NONE', #25340, #6328, #4394 ) ;
#90921=CIRCLE ( 'NONE', #36658, 0.1000000000000000472 ) ;
#90922=EDGE_CURVE ( 'NONE', #15358, #62185, #68821, .T. ) ;
#90923=DIRECTION ( 'NONE',  ( 0.000000000000000000, 0.000000000000000000, 1.000000000000000000 ) ) ;
#90924=AXIS2_PLACEMENT_3D ( 'NONE', #5400, #105549, #96347 ) ;
#90925=ORIENTED_EDGE ( 'NONE', *, *, #64024, .F. ) ;
#90926=CARTESIAN_POINT ( 'NONE',  ( 17.50000000000000000, 2.500000000000000000, 0.000000000000000000 ) ) ;
#90927=DIRECTION ( 'NONE',  ( 0.000000000000000000, 0.000000000000000000, -1.000000000000000000 ) ) ;
#90928=CARTESIAN_POINT ( 'NONE',  ( 9.149999999999916866, 2.500000000000000000, 5.902370205355745192 ) ) ;
#90929=DIRECTION ( 'NONE',  ( -0.000000000000000000, 1.000000000000000000, -0.000000000000000000 ) ) ;
#90930=ADVANCED_FACE ( 'NONE', ( #100418 ), #77230, .T. ) ;
#90931=ORIENTED_EDGE ( 'NONE', *, *, #20289, .T. ) ;
#90932=ORIENTED_EDGE ( 'NONE', *, *, #61238, .T. ) ;
#90933=VERTEX_POINT ( 'NONE', #91239 ) ;
#90934=DIRECTION ( 'NONE',  ( 0.000000000000000000, 0.000000000000000000, -1.000000000000000000 ) ) ;
#90935=EDGE_CURVE ( 'NONE', #118779, #33308, #4065, .T. ) ;
#90936=ADVANCED_FACE ( 'NONE', ( #99776 ), #87772, .T. ) ;
#90937=DIRECTION ( 'NONE',  ( -4.274815082592931898E-19, -0.9999939076577903929, -0.003490651415223739937 ) ) ;
#90938=EDGE_CURVE ( 'NONE', #9468, #14124, #38951, .T. ) ;
#90939=FACE_BOUND ( 'NONE', #2699, .T. ) ;
#90940=EDGE_CURVE ( 'NONE', #75204, #13568, #119093, .T. ) ;
#90941=LINE ( 'NONE', #59578, #53500 ) ;
#90942=AXIS2_PLACEMENT_3D ( 'NONE', #36893, #76813, #17876 ) ;
#90943=FACE_OUTER_BOUND ( 'NONE', #14612, .T. ) ;
#90944=CARTESIAN_POINT ( 'NONE',  ( -3.750000000000026201, 12.50000000000000000, 5.737276932171707422 ) ) ;
#90945=EDGE_CURVE ( 'NONE', #24882, #28910, #64798, .T. ) ;
#90946=CARTESIAN_POINT ( 'NONE',  ( -1.650000000000034772, 12.50000000000000000, 2.165063509461097713 ) ) ;
#90947=EDGE_CURVE ( 'NONE', #93321, #34505, #14605, .T. ) ;
#90948=CARTESIAN_POINT ( 'NONE',  ( 5.849999999999933920, 12.50000000000000000, -2.857883832488653741 ) ) ;
#90949=EDGE_CURVE ( 'NONE', #79994, #33468, #10101, .T. ) ;
#90950=CARTESIAN_POINT ( 'NONE',  ( 11.64999999999990621, 2.500000000000000000, -2.065063509461102065 ) ) ;
#90951=EDGE_LOOP ( 'NONE', ( #91394, #110182, #36782, #19874 ) ) ;
#90952=AXIS2_PLACEMENT_3D ( 'NONE', #113516, #21267, #23866 ) ;
#90953=PLANE ( 'NONE',  #84626 ) ;
#90955=EDGE_CURVE ( 'NONE', #120418, #72840, #35480, .T. ) ;
#90956=DIRECTION ( 'NONE',  ( 0.000000000000000000, 0.000000000000000000, 1.000000000000000000 ) ) ;
#90957=VERTEX_POINT ( 'NONE', #89303 ) ;
#90958=EDGE_LOOP ( 'NONE', ( #37365, #47967 ) ) ;
#90959=DIRECTION ( 'NONE',  ( -0.000000000000000000, -1.000000000000000000, -0.000000000000000000 ) ) ;
#90961=FACE_BOUND ( 'NONE', #55083, .T. ) ;
#90962=EDGE_CURVE ( 'NONE', #85218, #111831, #89941, .T. ) ;
#90963=CARTESIAN_POINT ( 'NONE',  ( 14.93814514904464197, -2.499999999999999556, -6.173787961026617310 ) ) ;
#90964=AXIS2_PLACEMENT_3D ( 'NONE', #1412, #59059, #21712 ) ;
#90965=DIRECTION ( 'NONE',  ( -0.000000000000000000, -1.000000000000000000, -0.000000000000000000 ) ) ;
#90966=CIRCLE ( 'NONE', #111897, 0.06509327318403745899 ) ;
#90967=ORIENTED_EDGE ( 'NONE', *, *, #13824, .T. ) ;
#90968=DIRECTION ( 'NONE',  ( 0.000000000000000000, 1.000000000000000000, 0.000000000000000000 ) ) ;
#90970=ORIENTED_EDGE ( 'NONE', *, *, #6701, .T. ) ;
#90971=CARTESIAN_POINT ( 'NONE',  ( -6.450000000000019718, 2.500000000000000000, -1.718653347947326049 ) ) ;
#90972=DIRECTION ( 'NONE',  ( 0.000000000000000000, 1.000000000000000000, 0.000000000000000000 ) ) ;
#90973=VECTOR ( 'NONE', #35737, 1000.000000000000000 ) ;
#90974=CIRCLE ( 'NONE', #72110, 0.06509327318403745899 ) ;
#90975=DIRECTION ( 'NONE',  ( 0.000000000000000000, 1.000000000000000000, 0.000000000000000000 ) ) ;
#90976=DIRECTION ( 'NONE',  ( 0.000000000000000000, 0.000000000000000000, 1.000000000000000000 ) ) ;
#90977=ORIENTED_EDGE ( 'NONE', *, *, #7037, .F. ) ;
#90978=DIRECTION ( 'NONE',  ( -0.000000000000000000, 1.000000000000000000, -0.000000000000000000 ) ) ;
#90979=DIRECTION ( 'NONE',  ( -4.274815082592931898E-19, -0.9999939076577903929, -0.003490651415223739937 ) ) ;
#90981=ORIENTED_EDGE ( 'NONE', *, *, #48853, .F. ) ;
#90982=EDGE_LOOP ( 'NONE', ( #74157, #112968, #23308, #39268 ) ) ;
#90983=CARTESIAN_POINT ( 'NONE',  ( 4.149999999999941735, 2.500000000000000000, -5.802370205355749988 ) ) ;
#90984=AXIS2_PLACEMENT_3D ( 'NONE', #104688, #23565, #103422 ) ;
#90985=ORIENTED_EDGE ( 'NONE', *, *, #96126, .T. ) ;
#90986=DIRECTION ( 'NONE',  ( 0.000000000000000000, 1.000000000000000000, 0.000000000000000000 ) ) ;
#90987=DIRECTION ( 'NONE',  ( 0.000000000000000000, 0.000000000000000000, 1.000000000000000000 ) ) ;
#90988=ADVANCED_FACE ( 'NONE', ( #61795 ), #129261, .T. ) ;
#90989=AXIS2_PLACEMENT_3D ( 'NONE', #317, #51403, #20641 ) ;
#90990=DIRECTION ( 'NONE',  ( 0.000000000000000000, 1.000000000000000000, 0.000000000000000000 ) ) ;
#90991=ORIENTED_EDGE ( 'NONE', *, *, #126862, .F. ) ;
#90992=CONICAL_SURFACE ( 'NONE', #9431, 0.09999999999999982514, 0.003490658503988666988 ) ;
#90993=DIRECTION ( 'NONE',  ( 0.000000000000000000, 1.000000000000000000, 0.000000000000000000 ) ) ;
#90994=EDGE_CURVE ( 'NONE', #125586, #118617, #27150, .T. ) ;
#90995=DIRECTION ( 'NONE',  ( 0.000000000000000000, -0.9999939076577903929, 0.003490651415223739937 ) ) ;
#90996=CARTESIAN_POINT ( 'NONE',  ( 9.599999999999914380, 2.500000000000000000, -3.537306695894649966 ) ) ;
#90998=LINE ( 'NONE', #41911, #3571 ) ;
#90999=CARTESIAN_POINT ( 'NONE',  ( 2.499999999999947153, 2.500000000000000000, -3.637306695894650055 ) ) ;
#91000=CARTESIAN_POINT ( 'NONE',  ( -11.25000000000000000, 2.500000000000000000, 7.188010851410848723 ) ) ;
#91001=EDGE_CURVE ( 'NONE', #22620, #67345, #43894, .T. ) ;
#91002=ORIENTED_EDGE ( 'NONE', *, *, #34707, .T. ) ;
#91003=CIRCLE ( 'NONE', #17833, 0.06509327318403745899 ) ;
#91004=ORIENTED_EDGE ( 'NONE', *, *, #43010, .T. ) ;
#91005=AXIS2_PLACEMENT_3D ( 'NONE', #13908, #63680, #125789 ) ;
#91006=FACE_OUTER_BOUND ( 'NONE', #124364, .T. ) ;
#91007=ORIENTED_EDGE ( 'NONE', *, *, #59248, .F. ) ;
#91008=DIRECTION ( 'NONE',  ( 0.000000000000000000, 0.000000000000000000, -1.000000000000000000 ) ) ;
#91009=AXIS2_PLACEMENT_3D ( 'NONE', #105060, #15382, #125992 ) ;
#91010=VERTEX_POINT ( 'NONE', #63066 ) ;
#91011=ORIENTED_EDGE ( 'NONE', *, *, #110709, .F. ) ;
#91012=VERTEX_POINT ( 'NONE', #121995 ) ;
#91013=DIRECTION ( 'NONE',  ( -0.000000000000000000, 1.000000000000000000, -0.000000000000000000 ) ) ;
#91014=ADVANCED_FACE ( 'NONE', ( #22522 ), #110757, .T. ) ;
#91015=AXIS2_PLACEMENT_3D ( 'NONE', #122130, #1684, #388 ) ;
#91016=CARTESIAN_POINT ( 'NONE',  ( -3.350000000000028511, 2.500000000000000000, 2.857883832488649301 ) ) ;
#91017=AXIS2_PLACEMENT_3D ( 'NONE', #59780, #61036, #99689 ) ;
#91018=CARTESIAN_POINT ( 'NONE',  ( 3.949999999999939782, 2.500000000000000000, 2.511473670974873507 ) ) ;
#91019=VECTOR ( 'NONE', #61061, 1000.000000000000000 ) ;
#91020=FACE_OUTER_BOUND ( 'NONE', #104329, .T. ) ;
#91021=DIRECTION ( 'NONE',  ( 0.000000000000000000, -0.000000000000000000, -1.000000000000000000 ) ) ;
#91022=CARTESIAN_POINT ( 'NONE',  ( 3.349999999999944578, 2.500000000000000000, -5.802370205355749988 ) ) ;
#91023=CIRCLE ( 'NONE', #65970, 0.1000000000000002554 ) ;
#91024=CARTESIAN_POINT ( 'NONE',  ( -13.94999999999998863, 12.50000000000000000, -1.818653347947323917 ) ) ;
#91025=DIRECTION ( 'NONE',  ( -4.274815082592931898E-19, -0.9999939076577903929, -0.003490651415223739937 ) ) ;
#91026=DIRECTION ( 'NONE',  ( -4.274815082592931898E-19, -0.9999939076577903929, -0.003490651415223739937 ) ) ;
#91027=ORIENTED_EDGE ( 'NONE', *, *, #40306, .F. ) ;
#91028=CARTESIAN_POINT ( 'NONE',  ( -4.150000000000027889, 2.500000000000000000, -6.495190528383302464 ) ) ;
#91029=ORIENTED_EDGE ( 'NONE', *, *, #111780, .T. ) ;
#91030=ORIENTED_EDGE ( 'NONE', *, *, #66726, .T. ) ;
#91031=DIRECTION ( 'NONE',  ( 0.000000000000000000, 0.000000000000000000, 1.000000000000000000 ) ) ;
#91032=VECTOR ( 'NONE', #98858, 1000.000000000000000 ) ;
#91033=DIRECTION ( 'NONE',  ( 0.000000000000000000, 0.000000000000000000, 1.000000000000000000 ) ) ;
#91034=ADVANCED_FACE ( 'NONE', ( #43448 ), #10421, .T. ) ;
#91035=LINE ( 'NONE', #98918, #60881 ) ;
#91036=DIRECTION ( 'NONE',  ( 0.000000000000000000, 1.000000000000000000, 0.000000000000000000 ) ) ;
#91037=DIRECTION ( 'NONE',  ( 0.000000000000000000, 0.000000000000000000, -1.000000000000000000 ) ) ;
#91038=DIRECTION ( 'NONE',  ( -0.000000000000000000, 1.000000000000000000, -0.000000000000000000 ) ) ;
#91039=ORIENTED_EDGE ( 'NONE', *, *, #111840, .T. ) ;
#91040=CIRCLE ( 'NONE', #80585, 0.06509327318403745899 ) ;
#91041=EDGE_CURVE ( 'NONE', #63523, #61895, #60620, .T. ) ;
#91042=VECTOR ( 'NONE', #87272, 1000.000000000000000 ) ;
#91043=CONICAL_SURFACE ( 'NONE', #68050, 0.09999999999999999167, 0.003490658503988666988 ) ;
#91044=ORIENTED_EDGE ( 'NONE', *, *, #55092, .F. ) ;
#91045=VERTEX_POINT ( 'NONE', #94445 ) ;
#91047=EDGE_LOOP ( 'NONE', ( #64596, #62205, #5726, #98618 ) ) ;
#91048=EDGE_CURVE ( 'NONE', #53990, #4275, #50152, .T. ) ;
#91049=ORIENTED_EDGE ( 'NONE', *, *, #112351, .F. ) ;
#91050=LINE ( 'NONE', #12481, #29403 ) ;
#91051=DIRECTION ( 'NONE',  ( -0.000000000000000000, 1.000000000000000000, -0.000000000000000000 ) ) ;
#91052=AXIS2_PLACEMENT_3D ( 'NONE', #125061, #15068, #47152 ) ;
#91053=DIRECTION ( 'NONE',  ( 0.000000000000000000, 1.000000000000000000, 0.000000000000000000 ) ) ;
#91054=DIRECTION ( 'NONE',  ( 0.000000000000000000, 1.000000000000000000, 0.000000000000000000 ) ) ;
#91055=CARTESIAN_POINT ( 'NONE',  ( 87.50000000000001421, -2.781865847474095155, 7.000342182495693066 ) ) ;
#91056=ORIENTED_EDGE ( 'NONE', *, *, #4997, .T. ) ;
#91057=DIRECTION ( 'NONE',  ( 0.000000000000000000, -0.000000000000000000, 1.000000000000000000 ) ) ;
#91058=LINE ( 'NONE', #1376, #93343 ) ;
#91059=EDGE_CURVE ( 'NONE', #100810, #38970, #8265, .T. ) ;
#91060=CARTESIAN_POINT ( 'NONE',  ( -7.100000000000018296, 2.500000000000000000, -4.430127018922202176 ) ) ;
#91061=FACE_OUTER_BOUND ( 'NONE', #78062, .T. ) ;
#91062=DIRECTION ( 'NONE',  ( 0.000000000000000000, 0.000000000000000000, 1.000000000000000000 ) ) ;
#91063=ORIENTED_EDGE ( 'NONE', *, *, #74650, .T. ) ;
#91064=AXIS2_PLACEMENT_3D ( 'NONE', #94482, #5458, #124610 ) ;
#91065=CIRCLE ( 'NONE', #55475, 0.1000000000000002554 ) ;
#91066=EDGE_LOOP ( 'NONE', ( #12830, #73888, #103109, #2152 ) ) ;
#91067=ORIENTED_EDGE ( 'NONE', *, *, #29059, .T. ) ;
#91068=DIRECTION ( 'NONE',  ( 0.000000000000000000, 0.000000000000000000, -1.000000000000000000 ) ) ;
#91069=ORIENTED_EDGE ( 'NONE', *, *, #122653, .F. ) ;
#91070=CARTESIAN_POINT ( 'NONE',  ( -0.8500000000000386136, 2.500000000000000000, 1.372243186433545370 ) ) ;
#91071=FACE_OUTER_BOUND ( 'NONE', #103175, .T. ) ;
#91072=ORIENTED_EDGE ( 'NONE', *, *, #105325, .F. ) ;
#91073=CARTESIAN_POINT ( 'NONE',  ( 12.29999999999990656, 2.500000000000000000, -4.676537180435977881 ) ) ;
#91074=DIRECTION ( 'NONE',  ( -0.000000000000000000, 1.000000000000000000, -0.000000000000000000 ) ) ;
#91075=DIRECTION ( 'NONE',  ( 0.000000000000000000, 0.000000000000000000, 1.000000000000000000 ) ) ;
#91076=AXIS2_PLACEMENT_3D ( 'NONE', #70580, #1192, #60142 ) ;
#91077=DIRECTION ( 'NONE',  ( 0.000000000000000000, 1.000000000000000000, 0.000000000000000000 ) ) ;
#91078=EDGE_CURVE ( 'NONE', #122576, #82140, #123293, .T. ) ;
#91079=AXIS2_PLACEMENT_3D ( 'NONE', #4833, #73579, #45434 ) ;
#91080=CARTESIAN_POINT ( 'NONE',  ( 2.499999999999983569, 12.50000000000000000, -2.276824562219559311E-15 ) ) ;
#91081=CIRCLE ( 'NONE', #109877, 0.1000000000000000056 ) ;
#91082=ORIENTED_EDGE ( 'NONE', *, *, #110575, .F. ) ;
#91084=ORIENTED_EDGE ( 'NONE', *, *, #94784, .F. ) ;
#91085=ADVANCED_FACE ( 'NONE', ( #91886 ), #72260, .T. ) ;
#91086=CARTESIAN_POINT ( 'NONE',  ( 65.34957883054167382, 3.515385111700535692, -5.621992225044548874 ) ) ;
#91087=CARTESIAN_POINT ( 'NONE',  ( 6.649999999999929301, 2.500000000000000000, 6.495190528383297135 ) ) ;
#91088=EDGE_CURVE ( 'NONE', #84285, #111183, #81445, .T. ) ;
#91089=DIRECTION ( 'NONE',  ( 0.000000000000000000, 1.000000000000000000, 0.000000000000000000 ) ) ;
#91090=DIRECTION ( 'NONE',  ( 0.000000000000000000, 0.000000000000000000, -1.000000000000000000 ) ) ;
#91091=VERTEX_POINT ( 'NONE', #33613 ) ;
#91092=ADVANCED_FACE ( 'NONE', ( #3506 ), #127504, .T. ) ;
#91093=CONICAL_SURFACE ( 'NONE', #40955, 0.1000000000000000472, 0.003490658503988666988 ) ;
#91094=ADVANCED_FACE ( 'NONE', ( #112819 ), #77322, .T. ) ;
#91095=ORIENTED_EDGE ( 'NONE', *, *, #120447, .F. ) ;
#91096=CARTESIAN_POINT ( 'NONE',  ( 1.449999999999951328, 2.500000000000000000, -1.918653347947326004 ) ) ;
#91097=DIRECTION ( 'NONE',  ( 0.000000000000000000, 1.000000000000000000, 0.000000000000000000 ) ) ;
#91098=ADVANCED_FACE ( 'NONE', ( #92521 ), #71067, .T. ) ;
#91099=DIRECTION ( 'NONE',  ( 0.000000000000000000, -0.000000000000000000, 1.000000000000000000 ) ) ;
#91100=ORIENTED_EDGE ( 'NONE', *, *, #15376, .T. ) ;
#91101=CIRCLE ( 'NONE', #11678, 2.000000000000000000 ) ;
#91102=AXIS2_PLACEMENT_3D ( 'NONE', #79879, #20320, #77942 ) ;
#91103=DIRECTION ( 'NONE',  ( -4.274815082592931898E-19, -0.9999939076577903929, -0.003490651415223739937 ) ) ;
#91104=CIRCLE ( 'NONE', #51329, 0.1000000000000000472 ) ;
#91105=EDGE_CURVE ( 'NONE', #97111, #108779, #79387, .T. ) ;
#91106=DIRECTION ( 'NONE',  ( -0.000000000000000000, -1.000000000000000000, -0.000000000000000000 ) ) ;
#91107=AXIS2_PLACEMENT_3D ( 'NONE', #37305, #117118, #127608 ) ;
#91108=VERTEX_POINT ( 'NONE', #59660 ) ;
#91109=DIRECTION ( 'NONE',  ( -4.274815082592931898E-19, -0.9999939076577903929, -0.003490651415223739937 ) ) ;
#91110=EDGE_LOOP ( 'NONE', ( #97320, #97348 ) ) ;
#91111=ADVANCED_FACE ( 'NONE', ( #2618 ), #109363, .T. ) ;
#91112=DIRECTION ( 'NONE',  ( 0.000000000000000000, 0.000000000000000000, 1.000000000000000000 ) ) ;
#91113=ORIENTED_EDGE ( 'NONE', *, *, #9857, .T. ) ;
#91114=ORIENTED_EDGE ( 'NONE', *, *, #65092, .T. ) ;
#91115=DIRECTION ( 'NONE',  ( 0.000000000000000000, 0.000000000000000000, 1.000000000000000000 ) ) ;
#91116=CARTESIAN_POINT ( 'NONE',  ( -3.950000000000028155, 2.500000000000000000, -6.741600689897077281 ) ) ;
#91117=EDGE_LOOP ( 'NONE', ( #109377, #47099 ) ) ;
#91118=ORIENTED_EDGE ( 'NONE', *, *, #9785, .F. ) ;
#91119=DIRECTION ( 'NONE',  ( 0.000000000000000000, -0.000000000000000000, 1.000000000000000000 ) ) ;
#91120=DIRECTION ( 'NONE',  ( 0.000000000000000000, 0.000000000000000000, 1.000000000000000000 ) ) ;
#91121=AXIS2_PLACEMENT_3D ( 'NONE', #65377, #126244, #76504 ) ;
#91122=EDGE_LOOP ( 'NONE', ( #5471, #14026, #102876, #12499 ) ) ;
#91125=CARTESIAN_POINT ( 'NONE',  ( 11.89999999999990798, 2.500000000000000000, 3.883716857408421319 ) ) ;
#91126=DIRECTION ( 'NONE',  ( -0.000000000000000000, -1.000000000000000000, -0.000000000000000000 ) ) ;
#91127=FACE_OUTER_BOUND ( 'NONE', #96446, .T. ) ;
#91128=DIRECTION ( 'NONE',  ( -0.000000000000000000, 1.000000000000000000, -0.000000000000000000 ) ) ;
#91129=CARTESIAN_POINT ( 'NONE',  ( -10.20000000000000462, 2.500000000000000000, 4.776537180435972196 ) ) ;
#91130=CIRCLE ( 'NONE', #109923, 0.06509327318403745899 ) ;
#91131=AXIS2_PLACEMENT_3D ( 'NONE', #15924, #95152, #55859 ) ;
#91132=ORIENTED_EDGE ( 'NONE', *, *, #112791, .F. ) ;
#91133=AXIS2_PLACEMENT_3D ( 'NONE', #7219, #86436, #126375 ) ;
#91134=VERTEX_POINT ( 'NONE', #100818 ) ;
#91135=DIRECTION ( 'NONE',  ( 0.000000000000000000, 1.000000000000000000, 0.000000000000000000 ) ) ;
#91136=ORIENTED_EDGE ( 'NONE', *, *, #44884, .F. ) ;
#91137=CARTESIAN_POINT ( 'NONE',  ( -9.150000000000009237, 12.50000000000000000, 2.792790559304612064 ) ) ;
#91138=LINE ( 'NONE', #89840, #99358 ) ;
#91139=CARTESIAN_POINT ( 'NONE',  ( 6.049999999999932321, 12.50000000000000000, 6.841600689897072485 ) ) ;
#91140=EDGE_LOOP ( 'NONE', ( #49582, #82033, #91162, #7621 ) ) ;
#91141=EDGE_LOOP ( 'NONE', ( #66329, #54359 ) ) ;
#91142=FACE_BOUND ( 'NONE', #103574, .T. ) ;
#91143=ORIENTED_EDGE ( 'NONE', *, *, #6487, .T. ) ;
#91144=DIRECTION ( 'NONE',  ( -0.000000000000000000, 1.000000000000000000, -0.000000000000000000 ) ) ;
#91145=CARTESIAN_POINT ( 'NONE',  ( -9.150000000000005684, 12.50000000000000000, 7.188010851410848723 ) ) ;
#91146=VECTOR ( 'NONE', #57466, 1000.000000000000000 ) ;
#91147=CARTESIAN_POINT ( 'NONE',  ( -3.350000000000028511, 2.500000000000000000, -1.572243186433550211 ) ) ;
#91148=LINE ( 'NONE', #62973, #80698 ) ;
#91149=EDGE_CURVE ( 'NONE', #39568, #18587, #70096, .T. ) ;
#91150=DIRECTION ( 'NONE',  ( 0.000000000000000000, 0.000000000000000000, -1.000000000000000000 ) ) ;
#91151=AXIS2_PLACEMENT_3D ( 'NONE', #92952, #124978, #47715 ) ;
#91152=AXIS2_PLACEMENT_3D ( 'NONE', #93094, #81337, #4043 ) ;
#91154=DIRECTION ( 'NONE',  ( 0.000000000000000000, 0.000000000000000000, -1.000000000000000000 ) ) ;
#91155=DIRECTION ( 'NONE',  ( 0.000000000000000000, 0.000000000000000000, 1.000000000000000000 ) ) ;
#91156=CARTESIAN_POINT ( 'NONE',  ( -3.100000000000028511, 2.500000000000000000, -0.3464101615137782364 ) ) ;
#91157=CARTESIAN_POINT ( 'NONE',  ( 11.64999999999990443, 2.500000000000000000, 1.372243186433545370 ) ) ;
#91158=CARTESIAN_POINT ( 'NONE',  ( -8.350000000000010303, 2.500000000000000000, 6.395190528383296602 ) ) ;
#91159=EDGE_CURVE ( 'NONE', #30305, #20100, #100199, .T. ) ;
#91160=EDGE_LOOP ( 'NONE', ( #125286, #68288, #117207, #121409 ) ) ;
#91161=ORIENTED_EDGE ( 'NONE', *, *, #67516, .T. ) ;
#91162=ORIENTED_EDGE ( 'NONE', *, *, #119224, .T. ) ;
#91163=ORIENTED_EDGE ( 'NONE', *, *, #39284, .F. ) ;
#91164=CARTESIAN_POINT ( 'NONE',  ( -1.250000000000037526, 12.50000000000000000, -5.867463478539787225 ) ) ;
#91165=CARTESIAN_POINT ( 'NONE',  ( 6.449999999999930012, 12.50000000000000000, 1.818653347947321475 ) ) ;
#91166=EDGE_LOOP ( 'NONE', ( #96114, #93301, #16465, #109955 ) ) ;
#91167=ORIENTED_EDGE ( 'NONE', *, *, #26814, .T. ) ;
#91168=ORIENTED_EDGE ( 'NONE', *, *, #113089, .T. ) ;
#91169=CARTESIAN_POINT ( 'NONE',  ( 9.799999999999913669, 12.50000000000000000, -3.983716857408426293 ) ) ;
#91170=DIRECTION ( 'NONE',  ( -0.000000000000000000, -1.000000000000000000, -0.000000000000000000 ) ) ;
#91172=DIRECTION ( 'NONE',  ( 0.000000000000000000, 0.000000000000000000, 1.000000000000000000 ) ) ;
#91173=DIRECTION ( 'NONE',  ( 0.000000000000000000, 0.000000000000000000, -1.000000000000000000 ) ) ;
#91174=DIRECTION ( 'NONE',  ( 0.000000000000000000, -0.000000000000000000, 1.000000000000000000 ) ) ;
#91175=CARTESIAN_POINT ( 'NONE',  ( -11.69999999999999929, 2.500000000000000000, -4.330127018922198978 ) ) ;
#91176=ORIENTED_EDGE ( 'NONE', *, *, #30600, .T. ) ;
#91177=DIRECTION ( 'NONE',  ( 0.000000000000000000, 0.000000000000000000, -1.000000000000000000 ) ) ;
#91178=VERTEX_POINT ( 'NONE', #19705 ) ;
#91179=AXIS2_PLACEMENT_3D ( 'NONE', #123819, #125744, #34181 ) ;
#91180=ORIENTED_EDGE ( 'NONE', *, *, #90614, .F. ) ;
#91181=ORIENTED_EDGE ( 'NONE', *, *, #490, .T. ) ;
#91182=CONICAL_SURFACE ( 'NONE', #97428, 0.09999999999999982514, 0.003490658503988666988 ) ;
#91183=CARTESIAN_POINT ( 'NONE',  ( -10.20000000000000284, 12.50000000000000000, -0.3464101615137782364 ) ) ;
#91184=ORIENTED_EDGE ( 'NONE', *, *, #86363, .F. ) ;
#91185=EDGE_LOOP ( 'NONE', ( #28321, #102703, #75860, #20648 ) ) ;
#91186=VERTEX_POINT ( 'NONE', #111959 ) ;
#91187=CONICAL_SURFACE ( 'NONE', #24569, 0.09999999999999999167, 0.003490658503988666988 ) ;
#91188=CONICAL_SURFACE ( 'NONE', #36821, 0.1000000000000002554, 0.003490658503988666988 ) ;
#91189=ADVANCED_FACE ( 'NONE', ( #32116 ), #51744, .T. ) ;
#91191=DIRECTION ( 'NONE',  ( 0.000000000000000000, 0.000000000000000000, 1.000000000000000000 ) ) ;
#91192=CARTESIAN_POINT ( 'NONE',  ( 12.49999999999990585, 2.500000000000000000, -4.922947341949753586 ) ) ;
#91193=CARTESIAN_POINT ( 'NONE',  ( -12.49999999999995737, 12.50000000000000000, 4.330127018922196314 ) ) ;
#91194=CARTESIAN_POINT ( 'NONE',  ( 5.199999999999931788, 12.50000000000000000, 4.676537180435972552 ) ) ;
#91195=LINE ( 'NONE', #50623, #17736 ) ;
#91196=AXIS2_PLACEMENT_3D ( 'NONE', #114079, #13281, #72237 ) ;
#91197=AXIS2_PLACEMENT_3D ( 'NONE', #16378, #75969, #33493 ) ;
#91198=EDGE_CURVE ( 'NONE', #69482, #60983, #70733, .T. ) ;
#91199=ORIENTED_EDGE ( 'NONE', *, *, #48114, .F. ) ;
#91200=DIRECTION ( 'NONE',  ( 0.000000000000000000, 0.000000000000000000, 1.000000000000000000 ) ) ;
#91201=CIRCLE ( 'NONE', #124565, 0.06509327318403745899 ) ;
#91202=EDGE_LOOP ( 'NONE', ( #101474, #22641 ) ) ;
#91203=DIRECTION ( 'NONE',  ( 0.000000000000000000, 0.000000000000000000, -1.000000000000000000 ) ) ;
#91204=DIRECTION ( 'NONE',  ( -4.274815082592931898E-19, -0.9999939076577903929, -0.003490651415223739937 ) ) ;
#91205=EDGE_LOOP ( 'NONE', ( #18213, #24901 ) ) ;
#91206=CARTESIAN_POINT ( 'NONE',  ( -8.350000000000013856, 2.500000000000000000, -6.495190528383297135 ) ) ;
#91207=EDGE_CURVE ( 'NONE', #122002, #90822, #72034, .T. ) ;
#91208=CARTESIAN_POINT ( 'NONE',  ( -11.84999999999999787, 2.500000000000000000, -6.048780366869523029 ) ) ;
#91209=ADVANCED_FACE ( 'NONE', ( #1981 ), #92297, .T. ) ;
#91210=ORIENTED_EDGE ( 'NONE', *, *, #14322, .T. ) ;
#91211=CARTESIAN_POINT ( 'NONE',  ( 7.899999999999924860, 2.500000000000000000, 3.537306695894645081 ) ) ;
#91212=EDGE_CURVE ( 'NONE', #119493, #58128, #102374, .T. ) ;
#91213=LINE ( 'NONE', #61768, #27944 ) ;
#91214=ORIENTED_EDGE ( 'NONE', *, *, #76454, .F. ) ;
#91215=VERTEX_POINT ( 'NONE', #89726 ) ;
#91216=CARTESIAN_POINT ( 'NONE',  ( 1.449999999999950440, 2.500000000000000000, 6.148780366869520009 ) ) ;
#91217=DIRECTION ( 'NONE',  ( -0.000000000000000000, -1.000000000000000000, -0.000000000000000000 ) ) ;
#91218=EDGE_CURVE ( 'NONE', #1029, #27988, #120479, .T. ) ;
#91220=AXIS2_PLACEMENT_3D ( 'NONE', #88217, #39181, #80379 ) ;
#91221=DIRECTION ( 'NONE',  ( -0.000000000000000000, 1.000000000000000000, -0.000000000000000000 ) ) ;
#91222=FACE_OUTER_BOUND ( 'NONE', #83594, .T. ) ;
#91223=ORIENTED_EDGE ( 'NONE', *, *, #93469, .T. ) ;
#91224=CIRCLE ( 'NONE', #80858, 0.1000000000000002554 ) ;
#91225=DIRECTION ( 'NONE',  ( 0.000000000000000000, 0.000000000000000000, 1.000000000000000000 ) ) ;
#91226=AXIS2_PLACEMENT_3D ( 'NONE', #5806, #33376, #85022 ) ;
#91227=AXIS2_PLACEMENT_3D ( 'NONE', #101926, #70520, #120912 ) ;
#91228=EDGE_LOOP ( 'NONE', ( #98461, #127806 ) ) ;
#91229=AXIS2_PLACEMENT_3D ( 'NONE', #109482, #118647, #129150 ) ;
#91230=DIRECTION ( 'NONE',  ( 0.000000000000000000, 0.000000000000000000, 1.000000000000000000 ) ) ;
#91231=FACE_OUTER_BOUND ( 'NONE', #93783, .T. ) ;
#91232=VECTOR ( 'NONE', #78036, 1000.000000000000000 ) ;
#91233=DIRECTION ( 'NONE',  ( 0.000000000000000000, 0.000000000000000000, 1.000000000000000000 ) ) ;
#91234=CARTESIAN_POINT ( 'NONE',  ( -1.700000000000034817, 2.500000000000000000, 0.09999999999999761857 ) ) ;
#91235=DIRECTION ( 'NONE',  ( 0.000000000000000000, -0.000000000000000000, 1.000000000000000000 ) ) ;
#91236=CARTESIAN_POINT ( 'NONE',  ( 8.349999999999923261, 2.500000000000000000, -6.495190528383302464 ) ) ;
#91237=LINE ( 'NONE', #53890, #78951 ) ;
#91238=EDGE_LOOP ( 'NONE', ( #52025, #19153, #76234, #85015 ) ) ;
#91239=CARTESIAN_POINT ( 'NONE',  ( 11.04999999999990656, 12.50000000000000000, 2.576566944158910744 ) ) ;
#91240=ADVANCED_FACE ( 'NONE', ( #21637 ), #11156, .T. ) ;
#91241=CIRCLE ( 'NONE', #72466, 0.09999999999999982514 ) ;
#91242=CIRCLE ( 'NONE', #126839, 0.06509327318403743123 ) ;
#91243=CARTESIAN_POINT ( 'NONE',  ( -1.050000000000038236, 2.500000000000000000, -6.148780366869526226 ) ) ;
#91244=FACE_OUTER_BOUND ( 'NONE', #72988, .T. ) ;
#91245=ORIENTED_EDGE ( 'NONE', *, *, #21326, .T. ) ;
#91246=EDGE_CURVE ( 'NONE', #69453, #57912, #81207, .T. ) ;
#91247=DIRECTION ( 'NONE',  ( -4.274815082592931898E-19, -0.9999939076577903929, -0.003490651415223739937 ) ) ;
#91248=VERTEX_POINT ( 'NONE', #50444 ) ;
#91249=ORIENTED_EDGE ( 'NONE', *, *, #98139, .F. ) ;
#91250=DIRECTION ( 'NONE',  ( -0.000000000000000000, -1.000000000000000000, -0.000000000000000000 ) ) ;
#91251=ADVANCED_FACE ( 'NONE', ( #61576 ), #16659, .T. ) ;
#91252=ORIENTED_EDGE ( 'NONE', *, *, #1380, .F. ) ;
#91253=CARTESIAN_POINT ( 'NONE',  ( 18.09676523921901037, -2.526776815558750222, -2.684906793687110049 ) ) ;
#91254=CARTESIAN_POINT ( 'NONE',  ( 12.09999999999990195, 12.50000000000000000, -2.276824562219559311E-15 ) ) ;
#91255=EDGE_CURVE ( 'NONE', #8978, #3854, #73123, .T. ) ;
#91256=EDGE_CURVE ( 'NONE', #31928, #62165, #45, .T. ) ;
#91257=ORIENTED_EDGE ( 'NONE', *, *, #86678, .F. ) ;
#91258=CARTESIAN_POINT ( 'NONE',  ( -11.64999999999999680, 12.50000000000000000, -2.099970236277060476 ) ) ;
#91259=EDGE_CURVE ( 'NONE', #129286, #38823, #50238, .T. ) ;
#91260=DIRECTION ( 'NONE',  ( 0.000000000000000000, 0.000000000000000000, 1.000000000000000000 ) ) ;
#91261=ORIENTED_EDGE ( 'NONE', *, *, #114105, .F. ) ;
#91262=EDGE_CURVE ( 'NONE', #1061, #93646, #83680, .T. ) ;
#91263=EDGE_CURVE ( 'NONE', #77376, #55889, #79487, .T. ) ;
#91264=AXIS2_PLACEMENT_3D ( 'NONE', #14980, #94217, #105332 ) ;
#91265=EDGE_LOOP ( 'NONE', ( #45116, #128913 ) ) ;
#91266=AXIS2_PLACEMENT_3D ( 'NONE', #76581, #98783, #77223 ) ;
#91267=ORIENTED_EDGE ( 'NONE', *, *, #109980, .F. ) ;
#91268=CARTESIAN_POINT ( 'NONE',  ( -7.900000000000014566, 12.50000000000000000, 0.6928203230275494784 ) ) ;
#91269=CARTESIAN_POINT ( 'NONE',  ( -6.900000000000019007, 12.50000000000000000, 0.3464101615137735735 ) ) ;
#91270=FACE_OUTER_BOUND ( 'NONE', #31008, .T. ) ;
#91271=FACE_BOUND ( 'NONE', #105692, .T. ) ;
#91272=ORIENTED_EDGE ( 'NONE', *, *, #47476, .F. ) ;
#91273=CARTESIAN_POINT ( 'NONE',  ( 7.899999999999923084, 2.500000000000000000, -0.6928203230275542523 ) ) ;
#91274=FACE_OUTER_BOUND ( 'NONE', #56328, .T. ) ;
#91275=ORIENTED_EDGE ( 'NONE', *, *, #59480, .T. ) ;
#91276=AXIS2_PLACEMENT_3D ( 'NONE', #105773, #106409, #19816 ) ;
#91277=DIRECTION ( 'NONE',  ( 0.000000000000000000, 0.000000000000000000, 1.000000000000000000 ) ) ;
#91278=DIRECTION ( 'NONE',  ( 0.000000000000000000, 0.000000000000000000, 1.000000000000000000 ) ) ;
#91279=FACE_OUTER_BOUND ( 'NONE', #38606, .T. ) ;
#91280=CARTESIAN_POINT ( 'NONE',  ( 2.499999999999947153, 12.50000000000000000, 3.637306695894644726 ) ) ;
#91281=DIRECTION ( 'NONE',  ( 0.000000000000000000, 0.000000000000000000, -1.000000000000000000 ) ) ;
#91282=DIRECTION ( 'NONE',  ( 0.000000000000000000, 1.000000000000000000, 0.000000000000000000 ) ) ;
#91283=FACE_OUTER_BOUND ( 'NONE', #106309, .T. ) ;
#91284=AXIS2_PLACEMENT_3D ( 'NONE', #98947, #60333, #110061 ) ;
#91285=AXIS2_PLACEMENT_3D ( 'NONE', #46502, #9170, #98828 ) ;
#91286=VECTOR ( 'NONE', #54315, 1000.000000000000000 ) ;
#91287=VERTEX_POINT ( 'NONE', #42583 ) ;
#91288=ORIENTED_EDGE ( 'NONE', *, *, #10270, .T. ) ;
#91289=EDGE_LOOP ( 'NONE', ( #75540, #88641 ) ) ;
#91290=ORIENTED_EDGE ( 'NONE', *, *, #112579, .F. ) ;
#91291=DIRECTION ( 'NONE',  ( 0.000000000000000000, 0.000000000000000000, 1.000000000000000000 ) ) ;
#91292=DIRECTION ( 'NONE',  ( -0.000000000000000000, 1.000000000000000000, -0.000000000000000000 ) ) ;
#91293=VERTEX_POINT ( 'NONE', #104060 ) ;
#91294=FACE_BOUND ( 'NONE', #106430, .T. ) ;
#91295=CARTESIAN_POINT ( 'NONE',  ( -9.150000000000011013, 2.500000000000000000, -5.902370205355745192 ) ) ;
#91296=DIRECTION ( 'NONE',  ( 0.000000000000000000, 0.000000000000000000, 1.000000000000000000 ) ) ;
#91297=DIRECTION ( 'NONE',  ( 0.000000000000000000, -0.9999939076577903929, 0.003490651415223739937 ) ) ;
#91298=DIRECTION ( 'NONE',  ( 0.000000000000000000, 0.000000000000000000, -1.000000000000000000 ) ) ;
#91299=CARTESIAN_POINT ( 'NONE',  ( -6.250000000000015987, 12.50000000000000000, 5.802370205355744659 ) ) ;
#91301=CARTESIAN_POINT ( 'NONE',  ( 9.149999999999920419, 2.500000000000000000, 2.757883832488649656 ) ) ;
#91302=FACE_OUTER_BOUND ( 'NONE', #72022, .T. ) ;
#91303=CARTESIAN_POINT ( 'NONE',  ( -9.550000000000006040, 2.500000000000000000, -2.265063509461101798 ) ) ;
#91304=AXIS2_PLACEMENT_3D ( 'NONE', #55421, #36445, #65875 ) ;
#91306=CIRCLE ( 'NONE', #47686, 0.06509327318403745899 ) ;
#91307=CIRCLE ( 'NONE', #83197, 0.06509327318403743123 ) ;
#91308=ORIENTED_EDGE ( 'NONE', *, *, #20357, .T. ) ;
#91310=ORIENTED_EDGE ( 'NONE', *, *, #62293, .F. ) ;
#91311=VECTOR ( 'NONE', #82749, 1000.000000000000000 ) ;
#91312=ORIENTED_EDGE ( 'NONE', *, *, #11322, .T. ) ;
#91313=VERTEX_POINT ( 'NONE', #75238 ) ;
#91314=EDGE_LOOP ( 'NONE', ( #1816, #71935 ) ) ;
#91315=CARTESIAN_POINT ( 'NONE',  ( 5.849999999999935696, 2.500000000000000000, -7.088010851410853519 ) ) ;
#91316=VERTEX_POINT ( 'NONE', #53032 ) ;
#91317=CIRCLE ( 'NONE', #34904, 0.1000000000000002554 ) ;
#91318=CIRCLE ( 'NONE', #55812, 0.1000000000000002554 ) ;
#91319=CONICAL_SURFACE ( 'NONE', #20309, 0.1000000000000002554, 0.003490658503988666988 ) ;
#91321=DIRECTION ( 'NONE',  ( 0.000000000000000000, -0.000000000000000000, 1.000000000000000000 ) ) ;
#91322=DIRECTION ( 'NONE',  ( 0.000000000000000000, 1.000000000000000000, 0.000000000000000000 ) ) ;
#91323=CARTESIAN_POINT ( 'NONE',  ( 5.649999999999936406, 2.500000000000000000, -6.941600689897077459 ) ) ;
#91324=CIRCLE ( 'NONE', #34912, 0.06509327318403745899 ) ;
#91325=ORIENTED_EDGE ( 'NONE', *, *, #93887, .T. ) ;
#91326=LINE ( 'NONE', #10799, #75590 ) ;
#91327=AXIS2_PLACEMENT_3D ( 'NONE', #9324, #21732, #19122 ) ;
#91328=VERTEX_POINT ( 'NONE', #94233 ) ;
#91329=AXIS2_PLACEMENT_3D ( 'NONE', #37737, #77637, #38396 ) ;
#91330=CONICAL_SURFACE ( 'NONE', #89278, 0.1000000000000002554, 0.003490658503988666988 ) ;
#91331=ORIENTED_EDGE ( 'NONE', *, *, #39020, .F. ) ;
#91332=LINE ( 'NONE', #122093, #17552 ) ;
#91333=CARTESIAN_POINT ( 'NONE',  ( -1.650000000000034328, 12.50000000000000000, -6.495190528383302464 ) ) ;
#91334=DIRECTION ( 'NONE',  ( -0.000000000000000000, -1.000000000000000000, -0.000000000000000000 ) ) ;
#91335=VERTEX_POINT ( 'NONE', #4534 ) ;
#91337=CARTESIAN_POINT ( 'NONE',  ( 1.699999999999951994, 12.50000000000000000, -4.330127018922201643 ) ) ;
#91338=DIRECTION ( 'NONE',  ( -4.274815082592931898E-19, -0.9999939076577903929, -0.003490651415223739937 ) ) ;
#91339=CARTESIAN_POINT ( 'NONE',  ( 12.89999999999990266, 2.500000000000000000, 5.022947341949748790 ) ) ;
#91340=CARTESIAN_POINT ( 'NONE',  ( 2.299999999999949640, 2.500000000000000000, -4.576537180435977348 ) ) ;
#91341=VERTEX_POINT ( 'NONE', #85056 ) ;
#91342=FACE_OUTER_BOUND ( 'NONE', #11144, .T. ) ;
#91343=AXIS2_PLACEMENT_3D ( 'NONE', #63302, #114334, #3735 ) ;
#91345=DIRECTION ( 'NONE',  ( 0.000000000000000000, 0.000000000000000000, -1.000000000000000000 ) ) ;
#91346=EDGE_CURVE ( 'NONE', #49349, #114386, #100407, .T. ) ;
#91347=EDGE_LOOP ( 'NONE', ( #31007, #37259, #2029, #122800 ) ) ;
#91348=DIRECTION ( 'NONE',  ( 0.000000000000000000, 0.000000000000000000, 1.000000000000000000 ) ) ;
#91349=CARTESIAN_POINT ( 'NONE',  ( 32.25969734032662473, -3.190781473932518875, 3.146220229225281440 ) ) ;
#91350=DIRECTION ( 'NONE',  ( 0.000000000000000000, -0.000000000000000000, 1.000000000000000000 ) ) ;
#91351=EDGE_CURVE ( 'NONE', #35123, #122362, #106657, .T. ) ;
#91352=DIRECTION ( 'NONE',  ( 0.000000000000000000, 1.000000000000000000, 0.000000000000000000 ) ) ;
#91353=ADVANCED_FACE ( 'NONE', ( #94882 ), #29306, .T. ) ;
#91354=ORIENTED_EDGE ( 'NONE', *, *, #112640, .F. ) ;
#91355=DIRECTION ( 'NONE',  ( 0.000000000000000000, 0.000000000000000000, 1.000000000000000000 ) ) ;
#91356=AXIS2_PLACEMENT_3D ( 'NONE', #37638, #24102, #77537 ) ;
#91357=EDGE_CURVE ( 'NONE', #81317, #29090, #123380, .T. ) ;
#91358=DIRECTION ( 'NONE',  ( 0.000000000000000000, 1.000000000000000000, 0.000000000000000000 ) ) ;
#91359=ORIENTED_EDGE ( 'NONE', *, *, #121628, .T. ) ;
#91360=EDGE_CURVE ( 'NONE', #39986, #54702, #43870, .T. ) ;
#91361=ORIENTED_EDGE ( 'NONE', *, *, #122252, .F. ) ;
#91362=EDGE_CURVE ( 'NONE', #96053, #84082, #35329, .T. ) ;
#91363=EDGE_LOOP ( 'NONE', ( #8573, #111380, #27365, #94476 ) ) ;
#91364=DIRECTION ( 'NONE',  ( 0.000000000000000000, 1.000000000000000000, 0.000000000000000000 ) ) ;
#91365=DIRECTION ( 'NONE',  ( 0.000000000000000000, 1.000000000000000000, 0.000000000000000000 ) ) ;
#91366=EDGE_CURVE ( 'NONE', #97899, #28983, #27232, .T. ) ;
#91367=CARTESIAN_POINT ( 'NONE',  ( -0.4500000000000397571, 12.50000000000000000, -2.099970236277064473 ) ) ;
#91368=FACE_OUTER_BOUND ( 'NONE', #65294, .T. ) ;
#91369=CONICAL_SURFACE ( 'NONE', #5666, 0.1000000000000002554, 0.003490658503988666988 ) ;
#91370=DIRECTION ( 'NONE',  ( 0.000000000000000000, 0.000000000000000000, 1.000000000000000000 ) ) ;
#91371=CIRCLE ( 'NONE', #60087, 0.06509327318403745899 ) ;
#91372=DIRECTION ( 'NONE',  ( 0.000000000000000000, 1.000000000000000000, 0.000000000000000000 ) ) ;
#91373=DIRECTION ( 'NONE',  ( 0.000000000000000000, 1.000000000000000000, 0.000000000000000000 ) ) ;
#91374=CARTESIAN_POINT ( 'NONE',  ( -1.850000000000033840, 2.500000000000000000, 2.411473670974873862 ) ) ;
#91375=AXIS2_PLACEMENT_3D ( 'NONE', #2335, #11530, #20075 ) ;
#91376=CIRCLE ( 'NONE', #34965, 0.06509327318403745899 ) ;
#91377=VECTOR ( 'NONE', #308, 1000.000000000000000 ) ;
#91378=ORIENTED_EDGE ( 'NONE', *, *, #98476, .F. ) ;
#91379=CARTESIAN_POINT ( 'NONE',  ( 8.949999999999921130, 2.500000000000000000, -6.841600689897078702 ) ) ;
#91380=CARTESIAN_POINT ( 'NONE',  ( -9.800000000000004263, 2.500000000000000000, -0.2464101615137783419 ) ) ;
#91381=DIRECTION ( 'NONE',  ( -0.000000000000000000, -1.000000000000000000, -0.000000000000000000 ) ) ;
#91382=DIRECTION ( 'NONE',  ( 0.000000000000000000, -0.000000000000000000, 1.000000000000000000 ) ) ;
#91383=ORIENTED_EDGE ( 'NONE', *, *, #99495, .F. ) ;
#91384=LINE ( 'NONE', #71757, #92701 ) ;
#91385=CARTESIAN_POINT ( 'NONE',  ( 1.449999999999951772, 2.500000000000000000, -6.248780366869526759 ) ) ;
#91386=LINE ( 'NONE', #1713, #2381 ) ;
#91387=EDGE_LOOP ( 'NONE', ( #17570, #65540, #44940, #61106 ) ) ;
#91388=EDGE_CURVE ( 'NONE', #25038, #9068, #123059, .T. ) ;
#91389=AXIS2_PLACEMENT_3D ( 'NONE', #102727, #72654, #3262 ) ;
#91390=ORIENTED_EDGE ( 'NONE', *, *, #8523, .T. ) ;
#91391=AXIS2_PLACEMENT_3D ( 'NONE', #92436, #2766, #10628 ) ;
#91392=DIRECTION ( 'NONE',  ( 0.000000000000000000, 0.000000000000000000, -1.000000000000000000 ) ) ;
#91393=AXIS2_PLACEMENT_3D ( 'NONE', #116688, #69520, #109455 ) ;
#91394=ORIENTED_EDGE ( 'NONE', *, *, #38682, .F. ) ;
#91395=ORIENTED_EDGE ( 'NONE', *, *, #9212, .F. ) ;
#91396=DIRECTION ( 'NONE',  ( 0.000000000000000000, 0.000000000000000000, 1.000000000000000000 ) ) ;
#91397=EDGE_CURVE ( 'NONE', #54474, #32010, #77415, .T. ) ;
#91398=ADVANCED_FACE ( 'NONE', ( #95536 ), #43974, .T. ) ;
#91399=CONICAL_SURFACE ( 'NONE', #116528, 0.09999999999999999167, 0.003490658503988666988 ) ;
#91400=DIRECTION ( 'NONE',  ( 0.000000000000000000, -0.9999939076577903929, 0.003490651415223739937 ) ) ;
#91401=DIRECTION ( 'NONE',  ( -4.274815082592931898E-19, -0.9999939076577903929, -0.003490651415223739937 ) ) ;
#91403=VECTOR ( 'NONE', #123483, 1000.000000000000000 ) ;
#91404=LINE ( 'NONE', #70476, #106455 ) ;
#91405=ORIENTED_EDGE ( 'NONE', *, *, #42678, .T. ) ;
#91407=DIRECTION ( 'NONE',  ( 0.000000000000000000, 0.000000000000000000, 1.000000000000000000 ) ) ;
#91408=ORIENTED_EDGE ( 'NONE', *, *, #3450, .T. ) ;
#91409=EDGE_CURVE ( 'NONE', #71314, #89603, #71148, .T. ) ;
#91410=DIRECTION ( 'NONE',  ( 0.000000000000000000, 1.000000000000000000, 0.000000000000000000 ) ) ;
#91411=CONICAL_SURFACE ( 'NONE', #7785, 0.09999999999999982514, 0.003490658503988666988 ) ;
#91412=EDGE_CURVE ( 'NONE', #113972, #19198, #114959, .T. ) ;
#91413=DIRECTION ( 'NONE',  ( -0.000000000000000000, 1.000000000000000000, -0.000000000000000000 ) ) ;
#91414=ADVANCED_FACE ( 'NONE', ( #93594 ), #62760, .T. ) ;
#91415=ORIENTED_EDGE ( 'NONE', *, *, #93046, .T. ) ;
#91416=EDGE_CURVE ( 'NONE', #20895, #123590, #2087, .T. ) ;
#91417=AXIS2_PLACEMENT_3D ( 'NONE', #93922, #74928, #86006 ) ;
#91418=AXIS2_PLACEMENT_3D ( 'NONE', #48482, #30633, #81007 ) ;
#91419=ADVANCED_FACE ( 'NONE', ( #117081 ), #7781, .T. ) ;
#91420=ORIENTED_EDGE ( 'NONE', *, *, #94787, .F. ) ;
#91421=ORIENTED_EDGE ( 'NONE', *, *, #106189, .F. ) ;
#91422=ORIENTED_EDGE ( 'NONE', *, *, #72772, .F. ) ;
#91423=DIRECTION ( 'NONE',  ( 0.000000000000000000, 1.000000000000000000, 0.000000000000000000 ) ) ;
#91424=CARTESIAN_POINT ( 'NONE',  ( 6.598553918452118694, 2.499999999999999112, 8.770211965177473701 ) ) ;
#91425=LINE ( 'NONE', #121507, #111050 ) ;
#91426=FACE_BOUND ( 'NONE', #83821, .T. ) ;
#91427=CARTESIAN_POINT ( 'NONE',  ( 4.149999999999939959, 2.500000000000000000, 2.857883832488649301 ) ) ;
#91429=ADVANCED_FACE ( 'NONE', ( #107277 ), #20979, .T. ) ;
#91430=DIRECTION ( 'NONE',  ( 0.000000000000000000, 0.000000000000000000, 1.000000000000000000 ) ) ;
#91431=LINE ( 'NONE', #71799, #8238 ) ;
#91432=DIRECTION ( 'NONE',  ( -0.000000000000000000, 1.000000000000000000, -0.000000000000000000 ) ) ;
#91433=CARTESIAN_POINT ( 'NONE',  ( -11.84999999999999787, 12.50000000000000000, -6.906693963081111498 ) ) ;
#91434=CONICAL_SURFACE ( 'NONE', #45487, 0.09999999999999982514, 0.003490658503988666988 ) ;
#91435=CARTESIAN_POINT ( 'NONE',  ( -10.45000000000000462, 2.500000000000000000, -2.165063509461097713 ) ) ;
#91436=DIRECTION ( 'NONE',  ( 0.000000000000000000, -0.000000000000000000, 1.000000000000000000 ) ) ;
#91437=VERTEX_POINT ( 'NONE', #68639 ) ;
#91438=VERTEX_POINT ( 'NONE', #77177 ) ;
#91439=ORIENTED_EDGE ( 'NONE', *, *, #34039, .F. ) ;
#91440=ORIENTED_EDGE ( 'NONE', *, *, #74412, .T. ) ;
#91441=EDGE_LOOP ( 'NONE', ( #57, #77765, #31059, #123803 ) ) ;
#91442=DIRECTION ( 'NONE',  ( 0.000000000000000000, 0.000000000000000000, 1.000000000000000000 ) ) ;
#91444=VERTEX_POINT ( 'NONE', #125614 ) ;
#91445=FACE_BOUND ( 'NONE', #44970, .T. ) ;
#91446=DIRECTION ( 'NONE',  ( -0.000000000000000000, -1.000000000000000000, -0.000000000000000000 ) ) ;
#91447=VECTOR ( 'NONE', #71529, 1000.000000000000000 ) ;
#91448=CONICAL_SURFACE ( 'NONE', #39255, 0.1000000000000002554, 0.003490658503988666988 ) ;
#91449=EDGE_LOOP ( 'NONE', ( #58554, #72612 ) ) ;
#91450=FACE_OUTER_BOUND ( 'NONE', #91238, .T. ) ;
#91451=PLANE ( 'NONE',  #91227 ) ;
#91452=FACE_OUTER_BOUND ( 'NONE', #187, .T. ) ;
#91453=DIRECTION ( 'NONE',  ( 0.000000000000000000, 0.000000000000000000, 1.000000000000000000 ) ) ;
#91454=EDGE_LOOP ( 'NONE', ( #27096, #81576 ) ) ;
#91455=CARTESIAN_POINT ( 'NONE',  ( -4.600000000000025402, 12.50000000000000000, 4.265033745738159077 ) ) ;
#91456=VECTOR ( 'NONE', #93505, 1000.000000000000000 ) ;
#91457=AXIS2_PLACEMENT_3D ( 'NONE', #123220, #31618, #83302 ) ;
#91458=EDGE_CURVE ( 'NONE', #53767, #65379, #27411, .T. ) ;
#91459=ORIENTED_EDGE ( 'NONE', *, *, #80122, .T. ) ;
#91460=ORIENTED_EDGE ( 'NONE', *, *, #59462, .F. ) ;
#91461=DIRECTION ( 'NONE',  ( 0.000000000000000000, 0.000000000000000000, -1.000000000000000000 ) ) ;
#91462=DIRECTION ( 'NONE',  ( 0.000000000000000000, 0.000000000000000000, 1.000000000000000000 ) ) ;
#91463=ORIENTED_EDGE ( 'NONE', *, *, #46156, .F. ) ;
#91464=LINE ( 'NONE', #34506, #83118 ) ;
#91465=CIRCLE ( 'NONE', #76805, 0.06509327318403745899 ) ;
#91466=AXIS2_PLACEMENT_3D ( 'NONE', #13851, #53782, #95009 ) ;
#91467=CARTESIAN_POINT ( 'NONE',  ( 12.29999999999990301, 12.50000000000000000, -0.2813168883297408329 ) ) ;
#91468=CARTESIAN_POINT ( 'NONE',  ( -7.900000000000011013, 12.50000000000000000, 5.088040615133786027 ) ) ;
#91469=DIRECTION ( 'NONE',  ( -0.000000000000000000, 1.000000000000000000, -0.000000000000000000 ) ) ;
#91471=VERTEX_POINT ( 'NONE', #98098 ) ;
#91472=EDGE_CURVE ( 'NONE', #63798, #59733, #7128, .T. ) ;
#91473=CARTESIAN_POINT ( 'NONE',  ( 5.799999999999934985, 2.500000000000000000, -4.330127018922201643 ) ) ;
#91474=ORIENTED_EDGE ( 'NONE', *, *, #127470, .T. ) ;
#91475=CARTESIAN_POINT ( 'NONE',  ( 3.349999999999943689, 2.500000000000000000, 1.572243186433545548 ) ) ;
#91476=AXIS2_PLACEMENT_3D ( 'NONE', #14654, #25133, #55254 ) ;
#91477=ORIENTED_EDGE ( 'NONE', *, *, #14336, .T. ) ;
#91478=DIRECTION ( 'NONE',  ( 0.000000000000000000, 0.000000000000000000, -1.000000000000000000 ) ) ;
#91479=EDGE_LOOP ( 'NONE', ( #121765, #5185, #19365, #26313 ) ) ;
#91480=CARTESIAN_POINT ( 'NONE',  ( -3.350000000000032507, 2.500000000000000000, -6.495190528383302464 ) ) ;
#91481=AXIS2_PLACEMENT_3D ( 'NONE', #98870, #117194, #7908 ) ;
#91483=LINE ( 'NONE', #41765, #88538 ) ;
#91484=DIRECTION ( 'NONE',  ( 0.000000000000000000, 0.000000000000000000, -1.000000000000000000 ) ) ;
#91485=DIRECTION ( 'NONE',  ( 0.000000000000000000, 1.000000000000000000, 0.000000000000000000 ) ) ;
#91486=CIRCLE ( 'NONE', #66348, 0.09999999999999982514 ) ;
#91487=ORIENTED_EDGE ( 'NONE', *, *, #39578, .F. ) ;
#91488=VECTOR ( 'NONE', #127710, 1000.000000000000000 ) ;
#91489=EDGE_LOOP ( 'NONE', ( #56549, #95481 ) ) ;
#91490=VERTEX_POINT ( 'NONE', #85699 ) ;
#91491=CARTESIAN_POINT ( 'NONE',  ( -0.6000000000000323963, 12.50000000000000000, 0.4115034346978133639 ) ) ;
#91492=AXIS2_PLACEMENT_3D ( 'NONE', #118113, #28467, #89944 ) ;
#91493=DIRECTION ( 'NONE',  ( -0.000000000000000000, 1.000000000000000000, -0.000000000000000000 ) ) ;
#91494=DIRECTION ( 'NONE',  ( 0.000000000000000000, 0.000000000000000000, 1.000000000000000000 ) ) ;
#91495=ORIENTED_EDGE ( 'NONE', *, *, #86045, .T. ) ;
#91496=ORIENTED_EDGE ( 'NONE', *, *, #44871, .T. ) ;
#91497=VERTEX_POINT ( 'NONE', #67320 ) ;
#91498=DIRECTION ( 'NONE',  ( 0.000000000000000000, 1.000000000000000000, 0.000000000000000000 ) ) ;
#91499=CONICAL_SURFACE ( 'NONE', #3764, 0.1000000000000002554, 0.003490658503988666988 ) ;
#91500=CIRCLE ( 'NONE', #85242, 0.06509327318403745899 ) ;
#91501=EDGE_LOOP ( 'NONE', ( #45890, #71245 ) ) ;
#91502=CARTESIAN_POINT ( 'NONE',  ( 7.099999999999926814, 2.500000000000000000, 0.09999999999999772959 ) ) ;
#91503=CARTESIAN_POINT ( 'NONE',  ( 10.84999999999990905, 2.500000000000000000, 2.757883832488649656 ) ) ;
#91504=CIRCLE ( 'NONE', #64310, 0.06509327318403745899 ) ;
#91505=EDGE_CURVE ( 'NONE', #22140, #7809, #47087, .T. ) ;
#91506=CARTESIAN_POINT ( 'NONE',  ( -11.44999999999999751, 2.500000000000000000, -6.841600689897074261 ) ) ;
#91507=DIRECTION ( 'NONE',  ( 0.000000000000000000, 0.000000000000000000, 1.000000000000000000 ) ) ;
#91508=CARTESIAN_POINT ( 'NONE',  ( 12.29999999999990479, 2.500000000000000000, -3.983716857408426293 ) ) ;
#91509=LINE ( 'NONE', #52238, #3255 ) ;
#91510=DIRECTION ( 'NONE',  ( 0.000000000000000000, -0.9999939076577903929, 0.003490651415223739937 ) ) ;
#91511=CIRCLE ( 'NONE', #122914, 0.06509327318403745899 ) ;
#91512=CARTESIAN_POINT ( 'NONE',  ( 0.4499999999999552136, 12.50000000000000000, 6.495190528383297135 ) ) ;
#91513=ADVANCED_FACE ( 'NONE', ( #57542 ), #41838, .T. ) ;
#91514=ORIENTED_EDGE ( 'NONE', *, *, #57832, .F. ) ;
#91515=DIRECTION ( 'NONE',  ( 0.000000000000000000, 1.000000000000000000, 0.000000000000000000 ) ) ;
#91516=CIRCLE ( 'NONE', #47611, 0.06509327318403745899 ) ;
#91517=CARTESIAN_POINT ( 'NONE',  ( 43.31961220463779938, -2.029667686306299235, 5.113275312221519542 ) ) ;
#91518=ADVANCED_FACE ( 'NONE', ( #38568 ), #85721, .T. ) ;
#91519=ORIENTED_EDGE ( 'NONE', *, *, #646, .F. ) ;
#91520=ADVANCED_FACE ( 'NONE', ( #58199 ), #110850, .T. ) ;
#91521=EDGE_LOOP ( 'NONE', ( #85689, #100727, #106138, #122157 ) ) ;
#91523=EDGE_CURVE ( 'NONE', #100782, #96782, #119184, .T. ) ;
#91525=DIRECTION ( 'NONE',  ( 0.000000000000000000, 0.000000000000000000, 1.000000000000000000 ) ) ;
#91526=EDGE_CURVE ( 'NONE', #113663, #123590, #75881, .T. ) ;
#91527=EDGE_CURVE ( 'NONE', #45295, #60915, #36628, .T. ) ;
#91528=CARTESIAN_POINT ( 'NONE',  ( -3.550000000000028244, 2.500000000000000000, 2.511473670974873507 ) ) ;
#91529=DIRECTION ( 'NONE',  ( 0.000000000000000000, 1.000000000000000000, 0.000000000000000000 ) ) ;
#91530=CARTESIAN_POINT ( 'NONE',  ( 12.04999999999990479, 12.50000000000000000, -6.495190528383302464 ) ) ;
#91531=DIRECTION ( 'NONE',  ( 0.000000000000000000, 0.000000000000000000, -1.000000000000000000 ) ) ;
#91532=FACE_OUTER_BOUND ( 'NONE', #31557, .T. ) ;
#91533=FACE_OUTER_BOUND ( 'NONE', #39429, .T. ) ;
#91534=EDGE_CURVE ( 'NONE', #61946, #18239, #73217, .T. ) ;
#91535=DIRECTION ( 'NONE',  ( 0.000000000000000000, 0.000000000000000000, 1.000000000000000000 ) ) ;
#91536=ADVANCED_FACE ( 'NONE', ( #18249 ), #118382, .T. ) ;
#91537=ORIENTED_EDGE ( 'NONE', *, *, #123318, .T. ) ;
#91539=ORIENTED_EDGE ( 'NONE', *, *, #11037, .T. ) ;
#91540=VERTEX_POINT ( 'NONE', #108746 ) ;
#91541=AXIS2_PLACEMENT_3D ( 'NONE', #80075, #70905, #120004 ) ;
#91542=ORIENTED_EDGE ( 'NONE', *, *, #39379, .T. ) ;
#91543=CARTESIAN_POINT ( 'NONE',  ( -8.550000000000009592, 12.50000000000000000, 6.776507416713035248 ) ) ;
#91544=DIRECTION ( 'NONE',  ( 0.000000000000000000, 0.000000000000000000, 1.000000000000000000 ) ) ;
#91545=ORIENTED_EDGE ( 'NONE', *, *, #44067, .F. ) ;
#91546=CIRCLE ( 'NONE', #39341, 0.06509327318403745899 ) ;
#91547=DIRECTION ( 'NONE',  ( 0.000000000000000000, 0.000000000000000000, -1.000000000000000000 ) ) ;
#91548=AXIS2_PLACEMENT_3D ( 'NONE', #127778, #118601, #49245 ) ;
#91549=LINE ( 'NONE', #19587, #113518 ) ;
#91550=DIRECTION ( 'NONE',  ( 0.000000000000000000, 1.000000000000000000, 0.000000000000000000 ) ) ;
#91551=CARTESIAN_POINT ( 'NONE',  ( 5.399999999999933742, 12.50000000000000000, -2.385244779468109755E-15 ) ) ;
#91552=ORIENTED_EDGE ( 'NONE', *, *, #38009, .T. ) ;
#91553=CARTESIAN_POINT ( 'NONE',  ( -7.900000000000011013, 2.500000000000000000, 4.922947341949748257 ) ) ;
#91554=CIRCLE ( 'NONE', #24658, 0.09999999999999999167 ) ;
#91555=FACE_OUTER_BOUND ( 'NONE', #110590, .T. ) ;
#91556=ORIENTED_EDGE ( 'NONE', *, *, #48222, .F. ) ;
#91557=AXIS2_PLACEMENT_3D ( 'NONE', #117887, #128391, #38731 ) ;
#91558=ORIENTED_EDGE ( 'NONE', *, *, #83308, .T. ) ;
#91559=ORIENTED_EDGE ( 'NONE', *, *, #37928, .T. ) ;
#91560=ORIENTED_EDGE ( 'NONE', *, *, #19227, .T. ) ;
#91561=DIRECTION ( 'NONE',  ( -0.000000000000000000, 1.000000000000000000, -0.000000000000000000 ) ) ;
#91562=DIRECTION ( 'NONE',  ( 0.000000000000000000, 0.000000000000000000, 1.000000000000000000 ) ) ;
#91563=LINE ( 'NONE', #23461, #60808 ) ;
#91564=ORIENTED_EDGE ( 'NONE', *, *, #40064, .T. ) ;
#91565=DIRECTION ( 'NONE',  ( -0.000000000000000000, -1.000000000000000000, -0.000000000000000000 ) ) ;
#91566=EDGE_LOOP ( 'NONE', ( #81567, #78397 ) ) ;
#91567=CONICAL_SURFACE ( 'NONE', #49729, 0.09999999999999982514, 0.003490658503988666988 ) ;
#91568=CARTESIAN_POINT ( 'NONE',  ( -7.300000000000016698, 2.500000000000000000, -4.576537180435978236 ) ) ;
#91569=FACE_OUTER_BOUND ( 'NONE', #70883, .T. ) ;
#91570=DIRECTION ( 'NONE',  ( -0.000000000000000000, -1.000000000000000000, -0.000000000000000000 ) ) ;
#91571=CARTESIAN_POINT ( 'NONE',  ( -2.499999999999996003, 2.500000000000000000, -4.430127018922202176 ) ) ;
#91572=EDGE_CURVE ( 'NONE', #25412, #53467, #33513, .T. ) ;
#91573=EDGE_CURVE ( 'NONE', #70439, #6072, #108106, .T. ) ;
#91574=EDGE_LOOP ( 'NONE', ( #57263, #36037, #75265, #50339 ) ) ;
#91575=CONICAL_SURFACE ( 'NONE', #16239, 0.1000000000000000472, 0.003490658503988666988 ) ;
#91576=ADVANCED_FACE ( 'NONE', ( #76722 ), #25252, .T. ) ;
#91578=EDGE_LOOP ( 'NONE', ( #42475, #3273 ) ) ;
#91579=ORIENTED_EDGE ( 'NONE', *, *, #48422, .T. ) ;
#91580=CARTESIAN_POINT ( 'NONE',  ( -8.150000000000012790, 12.50000000000000000, 2.511473670974873507 ) ) ;
#91581=CARTESIAN_POINT ( 'NONE',  ( -6.050000000000017586, 2.500000000000000000, 1.818653347947321475 ) ) ;
#91582=FACE_BOUND ( 'NONE', #101585, .T. ) ;
#91583=AXIS2_PLACEMENT_3D ( 'NONE', #118693, #110804, #61062 ) ;
#91584=CARTESIAN_POINT ( 'NONE',  ( 0.3999999999999555023, 2.500000000000000000, 4.230127018922196669 ) ) ;
#91585=LINE ( 'NONE', #61497, #63315 ) ;
#91586=AXIS2_PLACEMENT_3D ( 'NONE', #39995, #692, #79904 ) ;
#91587=ADVANCED_FACE ( 'NONE', ( #27597 ), #58387, .T. ) ;
#91588=DIRECTION ( 'NONE',  ( -0.000000000000000000, 1.000000000000000000, -0.000000000000000000 ) ) ;
#91589=AXIS2_PLACEMENT_3D ( 'NONE', #84643, #67557, #118608 ) ;
#91590=CARTESIAN_POINT ( 'NONE',  ( -4.076600168545496672E-14, 12.50000000000000000, -5.022947341949754119 ) ) ;
#91591=CONICAL_SURFACE ( 'NONE', #28912, 0.1000000000000002554, 0.003490658503988666988 ) ;
#91592=LINE ( 'NONE', #64063, #86373 ) ;
#91593=LINE ( 'NONE', #61506, #65721 ) ;
#91594=VERTEX_POINT ( 'NONE', #17113 ) ;
#91595=FACE_OUTER_BOUND ( 'NONE', #52608, .T. ) ;
#91596=CARTESIAN_POINT ( 'NONE',  ( 4.999999999999938716, 2.500000000000000000, -4.922947341949753586 ) ) ;
#91597=EDGE_LOOP ( 'NONE', ( #81169, #43660 ) ) ;
#91598=VERTEX_POINT ( 'NONE', #47271 ) ;
#91599=DIRECTION ( 'NONE',  ( 0.000000000000000000, 1.000000000000000000, 0.000000000000000000 ) ) ;
#91600=AXIS2_PLACEMENT_3D ( 'NONE', #7067, #126873, #37208 ) ;
#91601=DIRECTION ( 'NONE',  ( 0.000000000000000000, 0.000000000000000000, 1.000000000000000000 ) ) ;
#91602=ADVANCED_FACE ( 'NONE', ( #26985 ), #121414, .T. ) ;
#91603=FACE_BOUND ( 'NONE', #88243, .T. ) ;
#91604=DIRECTION ( 'NONE',  ( 0.000000000000000000, 1.000000000000000000, 0.000000000000000000 ) ) ;
#91605=AXIS2_PLACEMENT_3D ( 'NONE', #90870, #90208, #48536 ) ;
#91606=AXIS2_PLACEMENT_3D ( 'NONE', #69499, #19778, #90420 ) ;
#91607=VERTEX_POINT ( 'NONE', #66887 ) ;
#91608=CARTESIAN_POINT ( 'NONE',  ( 8.949999999999919353, 2.500000000000000000, -6.148780366869526226 ) ) ;
#91610=EDGE_LOOP ( 'NONE', ( #95741, #69457 ) ) ;
#91611=CARTESIAN_POINT ( 'NONE',  ( -13.14999999999999147, 2.500000000000000000, -1.718653347947323828 ) ) ;
#91612=EDGE_CURVE ( 'NONE', #85023, #106593, #108791, .T. ) ;
#91614=AXIS2_PLACEMENT_3D ( 'NONE', #24161, #73900, #42533 ) ;
#91615=CARTESIAN_POINT ( 'NONE',  ( 13.14999999999989733, 12.50000000000000000, -1.818653347947325916 ) ) ;
#91616=CARTESIAN_POINT ( 'NONE',  ( 1.449999999999949551, 2.500000000000000000, 6.841600689897072485 ) ) ;
#91617=ORIENTED_EDGE ( 'NONE', *, *, #105416, .T. ) ;
#91618=AXIS2_PLACEMENT_3D ( 'NONE', #91709, #104106, #1385 ) ;
#91619=CARTESIAN_POINT ( 'NONE',  ( -10.60000000000000320, 12.50000000000000000, -4.676537180435973440 ) ) ;
#91620=DIRECTION ( 'NONE',  ( -0.000000000000000000, -1.000000000000000000, -0.000000000000000000 ) ) ;
#91621=CONICAL_SURFACE ( 'NONE', #99946, 0.1000000000000000472, 0.003490658503988666988 ) ;
#91622=AXIS2_PLACEMENT_3D ( 'NONE', #5189, #34690, #27402 ) ;
#91623=DIRECTION ( 'NONE',  ( 0.000000000000000000, 0.000000000000000000, 1.000000000000000000 ) ) ;
#91624=VERTEX_POINT ( 'NONE', #48555 ) ;
#91625=ORIENTED_EDGE ( 'NONE', *, *, #72682, .F. ) ;
#91626=EDGE_CURVE ( 'NONE', #24362, #56014, #78670, .T. ) ;
#91627=DIRECTION ( 'NONE',  ( 0.000000000000000000, 0.000000000000000000, -1.000000000000000000 ) ) ;
#91628=AXIS2_PLACEMENT_3D ( 'NONE', #115956, #76680, #55742 ) ;
#91629=EDGE_LOOP ( 'NONE', ( #34856, #20835 ) ) ;
#91630=DIRECTION ( 'NONE',  ( 0.000000000000000000, 0.000000000000000000, -1.000000000000000000 ) ) ;
#91631=DIRECTION ( 'NONE',  ( 0.000000000000000000, 1.000000000000000000, 0.000000000000000000 ) ) ;
#91632=CIRCLE ( 'NONE', #33159, 0.06509327318403743123 ) ;
#91633=CIRCLE ( 'NONE', #16387, 0.09999999999999999167 ) ;
#91634=DIRECTION ( 'NONE',  ( 0.000000000000000000, -0.9999939076577903929, 0.003490651415223739937 ) ) ;
#91635=ORIENTED_EDGE ( 'NONE', *, *, #90188, .T. ) ;
#91636=DIRECTION ( 'NONE',  ( 0.000000000000000000, 0.000000000000000000, 1.000000000000000000 ) ) ;
#91637=CARTESIAN_POINT ( 'NONE',  ( 12.09999999999990550, 2.500000000000000000, 4.330127018922196314 ) ) ;
#91638=DIRECTION ( 'NONE',  ( 0.000000000000000000, 0.000000000000000000, 1.000000000000000000 ) ) ;
#91639=LINE ( 'NONE', #30811, #99817 ) ;
#91641=DIRECTION ( 'NONE',  ( 0.000000000000000000, 1.000000000000000000, 0.000000000000000000 ) ) ;
#91642=AXIS2_PLACEMENT_3D ( 'NONE', #75166, #3839, #35252 ) ;
#91643=ORIENTED_EDGE ( 'NONE', *, *, #106022, .T. ) ;
#91644=CONICAL_SURFACE ( 'NONE', #100063, 0.1000000000000002554, 0.003490658503988666988 ) ;
#91645=EDGE_LOOP ( 'NONE', ( #26691, #24636, #45544, #53855 ) ) ;
#91646=FACE_OUTER_BOUND ( 'NONE', #25138, .T. ) ;
#91647=VERTEX_POINT ( 'NONE', #87170 ) ;
#91649=ORIENTED_EDGE ( 'NONE', *, *, #124232, .T. ) ;
#91650=VERTEX_POINT ( 'NONE', #98282 ) ;
#91651=VERTEX_POINT ( 'NONE', #68175 ) ;
#91652=CARTESIAN_POINT ( 'NONE',  ( 8.549999999999918998, 12.50000000000000000, 6.906693963081109722 ) ) ;
#91653=CONICAL_SURFACE ( 'NONE', #89505, 0.1000000000000002554, 0.003490658503988666988 ) ;
#91654=CARTESIAN_POINT ( 'NONE',  ( 7.099999999999928590, 12.50000000000000000, -5.022947341949754119 ) ) ;
#91655=CARTESIAN_POINT ( 'NONE',  ( 3.349999999999944578, 12.50000000000000000, -1.472243186433550122 ) ) ;
#91656=EDGE_CURVE ( 'NONE', #78690, #14821, #25176, .T. ) ;
#91658=DIRECTION ( 'NONE',  ( 0.000000000000000000, 0.000000000000000000, 1.000000000000000000 ) ) ;
#91659=DIRECTION ( 'NONE',  ( 0.000000000000000000, 1.000000000000000000, 0.000000000000000000 ) ) ;
#91660=DIRECTION ( 'NONE',  ( 0.000000000000000000, 1.000000000000000000, 0.000000000000000000 ) ) ;
#91661=DIRECTION ( 'NONE',  ( 0.000000000000000000, -0.000000000000000000, 1.000000000000000000 ) ) ;
#91662=CIRCLE ( 'NONE', #35241, 0.1000000000000002554 ) ;
#91663=CARTESIAN_POINT ( 'NONE',  ( -10.65000000000000213, 2.500000000000000000, 2.511473670974873507 ) ) ;
#91664=DIRECTION ( 'NONE',  ( 0.000000000000000000, 1.000000000000000000, 0.000000000000000000 ) ) ;
#91665=EDGE_CURVE ( 'NONE', #15249, #70431, #117255, .T. ) ;
#91666=AXIS2_PLACEMENT_3D ( 'NONE', #111825, #41810, #92166 ) ;
#91667=VERTEX_POINT ( 'NONE', #8597 ) ;
#91669=DIRECTION ( 'NONE',  ( -4.274815082592931898E-19, -0.9999939076577903929, -0.003490651415223739937 ) ) ;
#91670=EDGE_CURVE ( 'NONE', #2963, #121075, #118567, .T. ) ;
#91671=ORIENTED_EDGE ( 'NONE', *, *, #67113, .F. ) ;
#91672=ADVANCED_FACE ( 'NONE', ( #67518 ), #67020, .T. ) ;
#91673=ORIENTED_EDGE ( 'NONE', *, *, #93893, .F. ) ;
#91674=EDGE_CURVE ( 'NONE', #51834, #585, #9271, .T. ) ;
#91675=FACE_OUTER_BOUND ( 'NONE', #124975, .T. ) ;
#91676=CARTESIAN_POINT ( 'NONE',  ( 10.19999999999991402, 2.500000000000000000, 0.3464101615137735735 ) ) ;
#91677=ADVANCED_FACE ( 'NONE', ( #129069 ), #87810, .T. ) ;
#91678=DIRECTION ( 'NONE',  ( -0.000000000000000000, 1.000000000000000000, -0.000000000000000000 ) ) ;
#91679=CARTESIAN_POINT ( 'NONE',  ( 11.64999999999990443, 2.500000000000000000, 1.472243186433545459 ) ) ;
#91680=CARTESIAN_POINT ( 'NONE',  ( 1.899999999999951283, 2.500000000000000000, -4.576537180435977348 ) ) ;
#91681=CARTESIAN_POINT ( 'NONE',  ( 2.499999999999983569, 2.500000000000000000, -4.430127018922202176 ) ) ;
#91682=EDGE_CURVE ( 'NONE', #45181, #73774, #33603, .T. ) ;
#91683=CARTESIAN_POINT ( 'NONE',  ( 5.599999999999934808, 12.50000000000000000, -3.983716857408426293 ) ) ;
#91685=ADVANCED_FACE ( 'NONE', ( #39402 ), #19747, .T. ) ;
#91686=AXIS2_PLACEMENT_3D ( 'NONE', #47205, #56362, #106117 ) ;
#91687=EDGE_CURVE ( 'NONE', #23602, #119523, #104680, .T. ) ;
#91688=EDGE_CURVE ( 'NONE', #126431, #65030, #91050, .T. ) ;
#91689=VERTEX_POINT ( 'NONE', #40691 ) ;
#91690=ADVANCED_FACE ( 'NONE', ( #92329 ), #31541, .T. ) ;
#91691=ORIENTED_EDGE ( 'NONE', *, *, #24132, .T. ) ;
#91692=CONICAL_SURFACE ( 'NONE', #51991, 0.09999999999999982514, 0.003490658503988666988 ) ;
#91693=ORIENTED_EDGE ( 'NONE', *, *, #43928, .F. ) ;
#91694=AXIS2_PLACEMENT_3D ( 'NONE', #32559, #109139, #119613 ) ;
#91695=EDGE_LOOP ( 'NONE', ( #115687, #114503, #17588, #116124 ) ) ;
#91696=EDGE_CURVE ( 'NONE', #39901, #114154, #115048, .T. ) ;
#91697=CARTESIAN_POINT ( 'NONE',  ( -1.900000000000034106, 12.50000000000000000, -3.918623584224389056 ) ) ;
#91698=DIRECTION ( 'NONE',  ( 0.000000000000000000, 0.000000000000000000, -1.000000000000000000 ) ) ;
#91699=CONICAL_SURFACE ( 'NONE', #22764, 0.09999999999999999167, 0.003490658503988666988 ) ;
#91700=CIRCLE ( 'NONE', #56178, 0.06509327318403745899 ) ;
#91701=CARTESIAN_POINT ( 'NONE',  ( -7.100000000000018296, 2.500000000000000000, -4.330127018922201643 ) ) ;
#91702=CARTESIAN_POINT ( 'NONE',  ( -3.350000000000028511, 2.500000000000000000, 1.372243186433545370 ) ) ;
#91703=CARTESIAN_POINT ( 'NONE',  ( 12.29999999999990479, 2.500000000000000000, 4.576537180435972019 ) ) ;
#91704=VERTEX_POINT ( 'NONE', #91697 ) ;
#91705=DIRECTION ( 'NONE',  ( -0.000000000000000000, 1.000000000000000000, -0.000000000000000000 ) ) ;
#91706=CARTESIAN_POINT ( 'NONE',  ( -7.700000000000012612, 2.500000000000000000, 4.676537180435972552 ) ) ;
#91707=DIRECTION ( 'NONE',  ( 0.000000000000000000, 0.000000000000000000, 1.000000000000000000 ) ) ;
#91708=DIRECTION ( 'NONE',  ( -0.000000000000000000, 1.000000000000000000, -0.000000000000000000 ) ) ;
#91709=CARTESIAN_POINT ( 'NONE',  ( 3.349999999999945466, 12.50000000000000000, -2.857883832488653741 ) ) ;
#91710=ORIENTED_EDGE ( 'NONE', *, *, #94040, .T. ) ;
#91711=ORIENTED_EDGE ( 'NONE', *, *, #108801, .F. ) ;
#91712=VERTEX_POINT ( 'NONE', #111306 ) ;
#91713=FACE_OUTER_BOUND ( 'NONE', #120129, .T. ) ;
#91714=ORIENTED_EDGE ( 'NONE', *, *, #55153, .T. ) ;
#91715=LINE ( 'NONE', #71411, #109375 ) ;
#91716=CARTESIAN_POINT ( 'NONE',  ( 13.29999999999989946, 2.500000000000000000, 0.09999999999999761857 ) ) ;
#91717=AXIS2_PLACEMENT_3D ( 'NONE', #79175, #39895, #39263 ) ;
#91718=CIRCLE ( 'NONE', #112652, 0.09999999999999982514 ) ;
#91719=CIRCLE ( 'NONE', #35297, 0.1000000000000002554 ) ;
#91720=ORIENTED_EDGE ( 'NONE', *, *, #23703, .T. ) ;
#91721=DIRECTION ( 'NONE',  ( 0.000000000000000000, 1.000000000000000000, 0.000000000000000000 ) ) ;
#91722=CARTESIAN_POINT ( 'NONE',  ( 3.549999999999943867, 2.500000000000000000, -1.818653347947326138 ) ) ;
#91723=FACE_OUTER_BOUND ( 'NONE', #121885, .T. ) ;
#91724=LINE ( 'NONE', #123122, #110327 ) ;
#91725=AXIS2_PLACEMENT_3D ( 'NONE', #11659, #10999, #100048 ) ;
#91726=ADVANCED_FACE ( 'NONE', ( #11187 ), #113007, .T. ) ;
#91727=CIRCLE ( 'NONE', #29055, 0.06509327318403745899 ) ;
#91728=CARTESIAN_POINT ( 'NONE',  ( 7.099999999999928590, 12.50000000000000000, 3.637306695894644726 ) ) ;
#91729=ADVANCED_FACE ( 'NONE', ( #62885 ), #100230, .T. ) ;
#91730=ORIENTED_EDGE ( 'NONE', *, *, #38142, .T. ) ;
#91731=VERTEX_POINT ( 'NONE', #79936 ) ;
#91732=CARTESIAN_POINT ( 'NONE',  ( -6.650000000000018119, 2.500000000000000000, -6.495190528383302464 ) ) ;
#91733=AXIS2_PLACEMENT_3D ( 'NONE', #17347, #76295, #8186 ) ;
#91734=CARTESIAN_POINT ( 'NONE',  ( -7.500000000000015099, 12.50000000000000000, -0.6928203230275541413 ) ) ;
#91735=ADVANCED_FACE ( 'NONE', ( #42616 ), #96264, .T. ) ;
#91736=CARTESIAN_POINT ( 'NONE',  ( 1.849999999999948130, 2.500000000000000000, 6.148780366869520009 ) ) ;
#91737=VERTEX_POINT ( 'NONE', #61607 ) ;
#91738=EDGE_CURVE ( 'NONE', #72025, #71464, #82535, .T. ) ;
#91739=ORIENTED_EDGE ( 'NONE', *, *, #42936, .F. ) ;
#91740=CARTESIAN_POINT ( 'NONE',  ( 8.149999999999923972, 2.500000000000000000, 1.818653347947321475 ) ) ;
#91741=DIRECTION ( 'NONE',  ( -0.000000000000000000, -1.000000000000000000, -0.000000000000000000 ) ) ;
#91742=DIRECTION ( 'NONE',  ( 0.000000000000000000, 1.000000000000000000, 0.000000000000000000 ) ) ;
#91744=ORIENTED_EDGE ( 'NONE', *, *, #20285, .F. ) ;
#91745=AXIS2_PLACEMENT_3D ( 'NONE', #58794, #9031, #88897 ) ;
#91746=DIRECTION ( 'NONE',  ( 0.000000000000000000, 0.000000000000000000, 1.000000000000000000 ) ) ;
#91747=DIRECTION ( 'NONE',  ( 0.000000000000000000, -0.9999939076577903929, 0.003490651415223739937 ) ) ;
#91748=VECTOR ( 'NONE', #127450, 1000.000000000000000 ) ;
#91749=EDGE_LOOP ( 'NONE', ( #66262, #92635, #115972, #128213 ) ) ;
#91750=CARTESIAN_POINT ( 'NONE',  ( -6.700000000000016165, 12.50000000000000000, 4.395220292106234439 ) ) ;
#91751=EDGE_LOOP ( 'NONE', ( #9107, #54848, #58050, #52422 ) ) ;
#91753=ORIENTED_EDGE ( 'NONE', *, *, #95399, .T. ) ;
#91754=CIRCLE ( 'NONE', #87542, 0.1000000000000002554 ) ;
#91755=CARTESIAN_POINT ( 'NONE',  ( 13.34999999999990017, 12.50000000000000000, 2.165063509461097713 ) ) ;
#91756=DIRECTION ( 'NONE',  ( 0.000000000000000000, 0.000000000000000000, -1.000000000000000000 ) ) ;
#91757=EDGE_LOOP ( 'NONE', ( #57693, #102746, #97944, #44820 ) ) ;
#91758=ORIENTED_EDGE ( 'NONE', *, *, #19265, .F. ) ;
#91759=DIRECTION ( 'NONE',  ( -0.000000000000000000, 1.000000000000000000, -0.000000000000000000 ) ) ;
#91761=VECTOR ( 'NONE', #47408, 1000.000000000000000 ) ;
#91763=EDGE_CURVE ( 'NONE', #54102, #118, #127671, .T. ) ;
#91767=CARTESIAN_POINT ( 'NONE',  ( 9.399999999999915090, 12.50000000000000000, -4.676537180435977881 ) ) ;
#91768=CARTESIAN_POINT ( 'NONE',  ( -2.900000000000029665, 2.500000000000000000, 4.430127018922196847 ) ) ;
#91769=CARTESIAN_POINT ( 'NONE',  ( 2.299999999999947864, 12.50000000000000000, 3.983716857408420964 ) ) ;
#91770=DIRECTION ( 'NONE',  ( 0.000000000000000000, 0.000000000000000000, -1.000000000000000000 ) ) ;
#91771=VECTOR ( 'NONE', #90015, 1000.000000000000000 ) ;
#91772=VERTEX_POINT ( 'NONE', #30219 ) ;
#91773=VERTEX_POINT ( 'NONE', #50478 ) ;
#91775=CIRCLE ( 'NONE', #81321, 0.06509327318403745899 ) ;
#91776=VECTOR ( 'NONE', #99485, 1000.000000000000000 ) ;
#91777=VERTEX_POINT ( 'NONE', #30860 ) ;
#91778=CARTESIAN_POINT ( 'NONE',  ( 6.649999999999928413, 12.50000000000000000, 2.792790559304612064 ) ) ;
#91779=DIRECTION ( 'NONE',  ( 0.000000000000000000, 0.000000000000000000, 1.000000000000000000 ) ) ;
#91780=EDGE_CURVE ( 'NONE', #85421, #9409, #37797, .T. ) ;
#91781=DIRECTION ( 'NONE',  ( 0.000000000000000000, -0.9999939076577903929, 0.003490651415223739937 ) ) ;
#91782=CIRCLE ( 'NONE', #79285, 0.06509327318403745899 ) ;
#91783=ORIENTED_EDGE ( 'NONE', *, *, #26133, .T. ) ;
#91784=VERTEX_POINT ( 'NONE', #122455 ) ;
#91785=FACE_BOUND ( 'NONE', #94070, .T. ) ;
#91786=ORIENTED_EDGE ( 'NONE', *, *, #99580, .F. ) ;
#91787=ADVANCED_FACE ( 'NONE', ( #726 ), #120515, .T. ) ;
#91788=CARTESIAN_POINT ( 'NONE',  ( 13.09999999999990195, 2.500000000000000000, 4.676537180435972552 ) ) ;
#91789=DIRECTION ( 'NONE',  ( -0.000000000000000000, 1.000000000000000000, -0.000000000000000000 ) ) ;
#91790=DIRECTION ( 'NONE',  ( 0.000000000000000000, -0.000000000000000000, 1.000000000000000000 ) ) ;
#91791=CIRCLE ( 'NONE', #108507, 0.1000000000000002554 ) ;
#91792=CIRCLE ( 'NONE', #4042, 0.09999999999999982514 ) ;
#91793=CARTESIAN_POINT ( 'NONE',  ( 10.84999999999990905, 2.500000000000000000, 2.957883832488649389 ) ) ;
#91794=FACE_OUTER_BOUND ( 'NONE', #105666, .T. ) ;
#91795=DIRECTION ( 'NONE',  ( 0.000000000000000000, 0.000000000000000000, -1.000000000000000000 ) ) ;
#91796=FACE_OUTER_BOUND ( 'NONE', #90569, .T. ) ;
#91798=EDGE_CURVE ( 'NONE', #11533, #86367, #6367, .T. ) ;
#91799=DIRECTION ( 'NONE',  ( 0.000000000000000000, 0.000000000000000000, 1.000000000000000000 ) ) ;
#91800=DIRECTION ( 'NONE',  ( -0.000000000000000000, -1.000000000000000000, -0.000000000000000000 ) ) ;
#91801=DIRECTION ( 'NONE',  ( 0.000000000000000000, 0.000000000000000000, -1.000000000000000000 ) ) ;
#91802=ORIENTED_EDGE ( 'NONE', *, *, #59633, .T. ) ;
#91803=ORIENTED_EDGE ( 'NONE', *, *, #15376, .F. ) ;
#91804=ORIENTED_EDGE ( 'NONE', *, *, #126536, .T. ) ;
#91805=CARTESIAN_POINT ( 'NONE',  ( 9.399999999999918643, 2.500000000000000000, -0.3464101615137782364 ) ) ;
#91806=EDGE_LOOP ( 'NONE', ( #24992, #12096, #89079, #2993 ) ) ;
#91807=FACE_OUTER_BOUND ( 'NONE', #35660, .T. ) ;
#91808=CARTESIAN_POINT ( 'NONE',  ( -3.749999999999991118, 12.50000000000000000, 2.165063509461097713 ) ) ;
#91809=VERTEX_POINT ( 'NONE', #110680 ) ;
#91810=ORIENTED_EDGE ( 'NONE', *, *, #16427, .F. ) ;
#91811=ORIENTED_EDGE ( 'NONE', *, *, #21326, .F. ) ;
#91812=DIRECTION ( 'NONE',  ( -0.000000000000000000, 1.000000000000000000, -0.000000000000000000 ) ) ;
#91813=AXIS2_PLACEMENT_3D ( 'NONE', #61469, #1875, #121647 ) ;
#91814=CIRCLE ( 'NONE', #75088, 0.06509327318403745899 ) ;
#91815=CARTESIAN_POINT ( 'NONE',  ( 7.949999999999925571, 2.500000000000000000, 2.065063509461097624 ) ) ;
#91816=SURFACE_STYLE_USAGE ( .BOTH. , #111439 ) ;
#91817=FACE_OUTER_BOUND ( 'NONE', #99306, .T. ) ;
#91818=CARTESIAN_POINT ( 'NONE',  ( 3.949999999999941558, 2.500000000000000000, -1.918653347947326004 ) ) ;
#91819=LINE ( 'NONE', #44655, #47677 ) ;
#91820=DIRECTION ( 'NONE',  ( 0.000000000000000000, 0.000000000000000000, 1.000000000000000000 ) ) ;
#91821=VERTEX_POINT ( 'NONE', #21015 ) ;
#91822=AXIS2_PLACEMENT_3D ( 'NONE', #7493, #47437, #127290 ) ;
#91823=VECTOR ( 'NONE', #6964, 1000.000000000000000 ) ;
#91824=CARTESIAN_POINT ( 'NONE',  ( 7.299999999999926104, 2.500000000000000000, -0.3464101615137782364 ) ) ;
#91825=ORIENTED_EDGE ( 'NONE', *, *, #54605, .T. ) ;
#91826=EDGE_CURVE ( 'NONE', #123530, #81523, #2010, .T. ) ;
#91827=AXIS2_PLACEMENT_3D ( 'NONE', #83765, #113213, #121749 ) ;
#91828=ORIENTED_EDGE ( 'NONE', *, *, #108089, .F. ) ;
#91830=CARTESIAN_POINT ( 'NONE',  ( 14.99999999999989164, 2.500000000000000000, 0.6928203230275494784 ) ) ;
#91831=EDGE_LOOP ( 'NONE', ( #12322, #15971, #101394, #39933 ) ) ;
#91833=EDGE_LOOP ( 'NONE', ( #22285, #3754, #90112, #13470 ) ) ;
#91834=ADVANCED_FACE ( 'NONE', ( #111988 ), #87947, .T. ) ;
#91835=ORIENTED_EDGE ( 'NONE', *, *, #49588, .F. ) ;
#91836=CIRCLE ( 'NONE', #108553, 0.1000000000000000472 ) ;
#91837=EDGE_CURVE ( 'NONE', #82761, #62966, #39876, .T. ) ;
#91838=AXIS2_PLACEMENT_3D ( 'NONE', #32339, #123896, #123265 ) ;
#91839=FACE_OUTER_BOUND ( 'NONE', #5269, .T. ) ;
#91840=DIRECTION ( 'NONE',  ( 0.000000000000000000, 0.000000000000000000, 1.000000000000000000 ) ) ;
#91841=DIRECTION ( 'NONE',  ( -4.274815082592931898E-19, -0.9999939076577903929, -0.003490651415223739937 ) ) ;
#91842=CARTESIAN_POINT ( 'NONE',  ( 6.249999999999930722, 12.50000000000000000, 7.188010851410848723 ) ) ;
#91843=EDGE_CURVE ( 'NONE', #20339, #60435, #45826, .T. ) ;
#91844=FACE_OUTER_BOUND ( 'NONE', #127100, .T. ) ;
#91845=EDGE_CURVE ( 'NONE', #20279, #78706, #3950, .T. ) ;
#91847=CARTESIAN_POINT ( 'NONE',  ( -6.700000000000019718, 2.500000000000000000, -2.385244779468109755E-15 ) ) ;
#91848=ORIENTED_EDGE ( 'NONE', *, *, #37363, .T. ) ;
#91849=DIRECTION ( 'NONE',  ( 0.000000000000000000, -0.9999939076577903929, 0.003490651415223739937 ) ) ;
#91850=EDGE_CURVE ( 'NONE', #59573, #113873, #71238, .T. ) ;
#91851=ORIENTED_EDGE ( 'NONE', *, *, #60211, .T. ) ;
#91852=CARTESIAN_POINT ( 'NONE',  ( -8.300000000000009592, 2.500000000000000000, 4.230127018922196669 ) ) ;
#91853=AXIS2_PLACEMENT_3D ( 'NONE', #15959, #17239, #55269 ) ;
#91854=EDGE_LOOP ( 'NONE', ( #16056, #10837, #28090, #125817 ) ) ;
#91855=CARTESIAN_POINT ( 'NONE',  ( 4.999999999999933387, 12.50000000000000000, 4.957854068765711553 ) ) ;
#91856=ADVANCED_FACE ( 'NONE', ( #35362 ), #44058, .T. ) ;
#91857=ORIENTED_EDGE ( 'NONE', *, *, #126370, .T. ) ;
#91858=EDGE_CURVE ( 'NONE', #102274, #46680, #60787, .T. ) ;
#91860=CARTESIAN_POINT ( 'NONE',  ( 11.84999999999990372, 2.500000000000000000, -6.048780366869526581 ) ) ;
#91861=VERTEX_POINT ( 'NONE', #55637 ) ;
#91864=LINE ( 'NONE', #2178, #125016 ) ;
#91865=CARTESIAN_POINT ( 'NONE',  ( -9.350000000000008527, 2.500000000000000000, -6.741600689897071952 ) ) ;
#91866=CARTESIAN_POINT ( 'NONE',  ( 11.24999999999991118, 2.500000000000000000, -2.857883832488653741 ) ) ;
#91867=CARTESIAN_POINT ( 'NONE',  ( -7.100000000000014744, 12.50000000000000000, 4.330127018922196314 ) ) ;
#91868=AXIS2_PLACEMENT_3D ( 'NONE', #10056, #1509, #41471 ) ;
#91869=CARTESIAN_POINT ( 'NONE',  ( 10.59999999999991260, 2.500000000000000000, 0.2464101615137735679 ) ) ;
#91870=ORIENTED_EDGE ( 'NONE', *, *, #95048, .T. ) ;
#91871=DIRECTION ( 'NONE',  ( 0.000000000000000000, 0.000000000000000000, 1.000000000000000000 ) ) ;
#91872=AXIS2_PLACEMENT_3D ( 'NONE', #108861, #8716, #27727 ) ;
#91873=ORIENTED_EDGE ( 'NONE', *, *, #54390, .F. ) ;
#91874=DIRECTION ( 'NONE',  ( 0.000000000000000000, -0.000000000000000000, 1.000000000000000000 ) ) ;
#91875=CARTESIAN_POINT ( 'NONE',  ( -2.050000000000033129, 2.500000000000000000, 2.265063509461097357 ) ) ;
#91876=AXIS2_PLACEMENT_3D ( 'NONE', #96673, #49546, #128763 ) ;
#91877=AXIS2_PLACEMENT_3D ( 'NONE', #105635, #66339, #15936 ) ;
#91878=DIRECTION ( 'NONE',  ( -0.000000000000000000, 1.000000000000000000, -0.000000000000000000 ) ) ;
#91879=CARTESIAN_POINT ( 'NONE',  ( 8.349999999999919709, 2.500000000000000000, 7.088010851410848190 ) ) ;
#91880=CARTESIAN_POINT ( 'NONE',  ( -9.350000000000006750, 12.50000000000000000, -1.818653347947325916 ) ) ;
#91881=DIRECTION ( 'NONE',  ( 0.000000000000000000, 0.000000000000000000, 1.000000000000000000 ) ) ;
#91882=DIRECTION ( 'NONE',  ( 0.000000000000000000, 0.000000000000000000, 1.000000000000000000 ) ) ;
#91883=ORIENTED_EDGE ( 'NONE', *, *, #75701, .F. ) ;
#91885=VECTOR ( 'NONE', #111351, 1000.000000000000000 ) ;
#91886=FACE_OUTER_BOUND ( 'NONE', #63896, .T. ) ;
#91887=EDGE_CURVE ( 'NONE', #96815, #49458, #111021, .T. ) ;
#91888=CARTESIAN_POINT ( 'NONE',  ( 13.09999999999990195, 12.50000000000000000, 4.741630453620009789 ) ) ;
#91889=DIRECTION ( 'NONE',  ( 0.000000000000000000, 0.000000000000000000, -1.000000000000000000 ) ) ;
#91890=EDGE_CURVE ( 'NONE', #54921, #103269, #73989, .T. ) ;
#91892=ORIENTED_EDGE ( 'NONE', *, *, #72327, .T. ) ;
#91893=CARTESIAN_POINT ( 'NONE',  ( 5.649999999999936406, 12.50000000000000000, -6.776507416713039689 ) ) ;
#91894=ORIENTED_EDGE ( 'NONE', *, *, #47474, .F. ) ;
#91895=ORIENTED_EDGE ( 'NONE', *, *, #66107, .F. ) ;
#91896=DIRECTION ( 'NONE',  ( 0.000000000000000000, 0.000000000000000000, 1.000000000000000000 ) ) ;
#91897=VECTOR ( 'NONE', #36257, 1000.000000000000000 ) ;
#91898=ORIENTED_EDGE ( 'NONE', *, *, #76769, .F. ) ;
#91899=CARTESIAN_POINT ( 'NONE',  ( -6.250000000000021316, 12.50000000000000000, -5.867463478539787225 ) ) ;
#91900=LINE ( 'NONE', #42157, #59198 ) ;
#91901=DIRECTION ( 'NONE',  ( 0.000000000000000000, 0.000000000000000000, 1.000000000000000000 ) ) ;
#91902=ORIENTED_EDGE ( 'NONE', *, *, #24505, .F. ) ;
#91903=AXIS2_PLACEMENT_3D ( 'NONE', #83362, #53895, #123279 ) ;
#91904=FACE_OUTER_BOUND ( 'NONE', #37648, .T. ) ;
#91905=CIRCLE ( 'NONE', #108619, 0.09999999999999982514 ) ;
#91906=DIRECTION ( 'NONE',  ( -0.000000000000000000, -1.000000000000000000, -0.000000000000000000 ) ) ;
#91907=CIRCLE ( 'NONE', #39615, 0.1000000000000002554 ) ;
#91908=VERTEX_POINT ( 'NONE', #64804 ) ;
#91909=AXIS2_PLACEMENT_3D ( 'NONE', #92002, #94568, #24550 ) ;
#91910=CIRCLE ( 'NONE', #37640, 0.06509327318403745899 ) ;
#91911=ORIENTED_EDGE ( 'NONE', *, *, #110806, .T. ) ;
#91912=ORIENTED_EDGE ( 'NONE', *, *, #30549, .T. ) ;
#91913=PLANE ( 'NONE',  #102824 ) ;
#91914=DIRECTION ( 'NONE',  ( 0.000000000000000000, -0.000000000000000000, 1.000000000000000000 ) ) ;
#91915=CARTESIAN_POINT ( 'NONE',  ( 2.699999999999947331, 2.500000000000000000, -4.576537180435978236 ) ) ;
#91916=FACE_BOUND ( 'NONE', #94533, .T. ) ;
#91917=EDGE_LOOP ( 'NONE', ( #91214, #55576 ) ) ;
#91918=VECTOR ( 'NONE', #49925, 1000.000000000000000 ) ;
#91919=CARTESIAN_POINT ( 'NONE',  ( 7.699999999999923794, 2.500000000000000000, 4.676537180435972552 ) ) ;
#91920=DIRECTION ( 'NONE',  ( 0.000000000000000000, 0.000000000000000000, 1.000000000000000000 ) ) ;
#91921=EDGE_LOOP ( 'NONE', ( #12099, #33551 ) ) ;
#91922=AXIS2_PLACEMENT_3D ( 'NONE', #112807, #23129, #13293 ) ;
#91923=DIRECTION ( 'NONE',  ( 0.000000000000000000, 1.000000000000000000, 0.000000000000000000 ) ) ;
#91924=ADVANCED_FACE ( 'NONE', ( #36005 ), #73384, .T. ) ;
#91925=FACE_OUTER_BOUND ( 'NONE', #59967, .T. ) ;
#91926=AXIS2_PLACEMENT_3D ( 'NONE', #53908, #14601, #124584 ) ;
#91927=CARTESIAN_POINT ( 'NONE',  ( -9.600000000000008527, 12.50000000000000000, 4.330127018922196314 ) ) ;
#91928=LINE ( 'NONE', #53304, #59678 ) ;
#91930=DIRECTION ( 'NONE',  ( 0.000000000000000000, -0.000000000000000000, 1.000000000000000000 ) ) ;
#91931=CARTESIAN_POINT ( 'NONE',  ( 10.19999999999991225, 2.500000000000000000, 3.983716857408420076 ) ) ;
#91932=VECTOR ( 'NONE', #24279, 1000.000000000000000 ) ;
#91933=EDGE_CURVE ( 'NONE', #115197, #28423, #75913, .T. ) ;
#91934=EDGE_LOOP ( 'NONE', ( #31044, #31410 ) ) ;
#91935=ORIENTED_EDGE ( 'NONE', *, *, #39860, .F. ) ;
#91936=ORIENTED_EDGE ( 'NONE', *, *, #5337, .F. ) ;
#91937=VERTEX_POINT ( 'NONE', #93630 ) ;
#91938=CONICAL_SURFACE ( 'NONE', #16613, 0.1000000000000000472, 0.003490658503988666988 ) ;
#91939=DIRECTION ( 'NONE',  ( 0.000000000000000000, 0.000000000000000000, -1.000000000000000000 ) ) ;
#91940=ADVANCED_FACE ( 'NONE', ( #92995 ), #104717, .T. ) ;
#91942=ORIENTED_EDGE ( 'NONE', *, *, #44430, .F. ) ;
#91943=FACE_BOUND ( 'NONE', #102300, .T. ) ;
#91944=EDGE_CURVE ( 'NONE', #101605, #12823, #64159, .T. ) ;
#91945=CARTESIAN_POINT ( 'NONE',  ( -8.350000000000012079, 2.500000000000000000, 1.472243186433545459 ) ) ;
#91946=DIRECTION ( 'NONE',  ( 0.000000000000000000, 0.000000000000000000, -1.000000000000000000 ) ) ;
#91947=CARTESIAN_POINT ( 'NONE',  ( -8.350000000000008527, 12.50000000000000000, 5.802370205355744659 ) ) ;
#91948=DIRECTION ( 'NONE',  ( 0.000000000000000000, 0.000000000000000000, 1.000000000000000000 ) ) ;
#91949=DIRECTION ( 'NONE',  ( 0.000000000000000000, 0.000000000000000000, -1.000000000000000000 ) ) ;
#91951=CARTESIAN_POINT ( 'NONE',  ( -7.300000000000016698, 12.50000000000000000, -4.676537180435978769 ) ) ;
#91952=DIRECTION ( 'NONE',  ( 0.000000000000000000, 0.000000000000000000, 1.000000000000000000 ) ) ;
#91953=EDGE_CURVE ( 'NONE', #122362, #35123, #88031, .T. ) ;
#91954=CARTESIAN_POINT ( 'NONE',  ( -4.600000000000024514, 2.500000000000000000, 5.022947341949748790 ) ) ;
#91955=ORIENTED_EDGE ( 'NONE', *, *, #68212, .T. ) ;
#91956=ORIENTED_EDGE ( 'NONE', *, *, #28841, .T. ) ;
#91957=EDGE_LOOP ( 'NONE', ( #20230, #69470, #118356, #8082 ) ) ;
#91958=VERTEX_POINT ( 'NONE', #74628 ) ;
#91959=ORIENTED_EDGE ( 'NONE', *, *, #73435, .F. ) ;
#91960=ORIENTED_EDGE ( 'NONE', *, *, #9375, .T. ) ;
#91961=CARTESIAN_POINT ( 'NONE',  ( -4.150000000000025224, 12.50000000000000000, 5.802370205355744659 ) ) ;
#91962=AXIS2_PLACEMENT_3D ( 'NONE', #27396, #67309, #35955 ) ;
#91963=VERTEX_POINT ( 'NONE', #34072 ) ;
#91964=ORIENTED_EDGE ( 'NONE', *, *, #50410, .F. ) ;
#91965=AXIS2_PLACEMENT_3D ( 'NONE', #107660, #17974, #116168 ) ;
#91966=FACE_OUTER_BOUND ( 'NONE', #104985, .T. ) ;
#91967=CIRCLE ( 'NONE', #71041, 0.06509327318403745899 ) ;
#91968=DIRECTION ( 'NONE',  ( 0.000000000000000000, 0.000000000000000000, -1.000000000000000000 ) ) ;
#91970=PLANE ( 'NONE',  #42590 ) ;
#91971=ORIENTED_EDGE ( 'NONE', *, *, #53531, .T. ) ;
#91972=CARTESIAN_POINT ( 'NONE',  ( 12.49999999999990585, 12.50000000000000000, -5.022947341949754119 ) ) ;
#91973=AXIS2_PLACEMENT_3D ( 'NONE', #7331, #106817, #26354 ) ;
#91974=ORIENTED_EDGE ( 'NONE', *, *, #125179, .T. ) ;
#91975=ADVANCED_FACE ( 'NONE', ( #125018 ), #6455, .T. ) ;
#91976=EDGE_LOOP ( 'NONE', ( #128949, #54940 ) ) ;
#91977=PLANE ( 'NONE',  #86515 ) ;
#91978=CARTESIAN_POINT ( 'NONE',  ( -2.100000000000033840, 2.500000000000000000, 3.637306695894644726 ) ) ;
#91979=EDGE_CURVE ( 'NONE', #40490, #124385, #25350, .T. ) ;
#91980=VERTEX_POINT ( 'NONE', #15033 ) ;
#91981=EDGE_LOOP ( 'NONE', ( #74142, #48596, #11694, #36247 ) ) ;
#91982=EDGE_CURVE ( 'NONE', #24753, #43343, #67096, .T. ) ;
#91983=LINE ( 'NONE', #72359, #23403 ) ;
#91984=DIRECTION ( 'NONE',  ( 0.000000000000000000, 0.000000000000000000, -1.000000000000000000 ) ) ;
#91985=DIRECTION ( 'NONE',  ( 0.000000000000000000, 0.000000000000000000, 1.000000000000000000 ) ) ;
#91986=FACE_OUTER_BOUND ( 'NONE', #103944, .T. ) ;
#91987=ADVANCED_FACE ( 'NONE', ( #98774 ), #107309, .T. ) ;
#91988=EDGE_CURVE ( 'NONE', #27272, #75731, #106827, .T. ) ;
#91989=DIRECTION ( 'NONE',  ( -4.274815082592931898E-19, -0.9999939076577903929, -0.003490651415223739937 ) ) ;
#91990=ADVANCED_FACE ( 'NONE', ( #47120 ), #6495, .T. ) ;
#91991=EDGE_CURVE ( 'NONE', #45160, #47559, #81784, .T. ) ;
#91992=ORIENTED_EDGE ( 'NONE', *, *, #98565, .T. ) ;
#91993=CARTESIAN_POINT ( 'NONE',  ( 13.91976764350727080, -2.500000000000000888, 6.779443706236988554 ) ) ;
#91994=VECTOR ( 'NONE', #108569, 1000.000000000000000 ) ;
#91995=AXIS2_PLACEMENT_3D ( 'NONE', #99045, #38196, #97107 ) ;
#91996=ORIENTED_EDGE ( 'NONE', *, *, #90200, .T. ) ;
#91997=CARTESIAN_POINT ( 'NONE',  ( -6.450000000000019718, 2.500000000000000000, -6.148780366869526226 ) ) ;
#91998=EDGE_CURVE ( 'NONE', #53510, #108831, #10674, .T. ) ;
#91999=CARTESIAN_POINT ( 'NONE',  ( 65.38812792108305416, -3.824344329442378676, 5.305601465418086526 ) ) ;
#92000=DIRECTION ( 'NONE',  ( -4.274815082592931898E-19, -0.9999939076577903929, -0.003490651415223739937 ) ) ;
#92001=DIRECTION ( 'NONE',  ( 0.000000000000000000, 1.000000000000000000, 0.000000000000000000 ) ) ;
#92002=CARTESIAN_POINT ( 'NONE',  ( 6.649999999999927525, 2.500000000000000000, 2.165063509461097713 ) ) ;
#92003=ORIENTED_EDGE ( 'NONE', *, *, #27937, .F. ) ;
#92004=CIRCLE ( 'NONE', #35575, 0.1000000000000002554 ) ;
#92005=EDGE_CURVE ( 'NONE', #102522, #93617, #44150, .T. ) ;
#92006=DIRECTION ( 'NONE',  ( -0.000000000000000000, 1.000000000000000000, -0.000000000000000000 ) ) ;
#92007=DIRECTION ( 'NONE',  ( 0.000000000000000000, -0.000000000000000000, 1.000000000000000000 ) ) ;
#92008=EDGE_LOOP ( 'NONE', ( #92481, #38127, #92603, #13898 ) ) ;
#92009=VERTEX_POINT ( 'NONE', #56273 ) ;
#92010=ORIENTED_EDGE ( 'NONE', *, *, #99043, .T. ) ;
#92011=DIRECTION ( 'NONE',  ( -0.000000000000000000, -1.000000000000000000, -0.000000000000000000 ) ) ;
#92012=DIRECTION ( 'NONE',  ( -4.274815082592931898E-19, -0.9999939076577903929, -0.003490651415223739937 ) ) ;
#92013=DIRECTION ( 'NONE',  ( -0.000000000000000000, -1.000000000000000000, -0.000000000000000000 ) ) ;
#92014=AXIS2_PLACEMENT_3D ( 'NONE', #23664, #4009, #43957 ) ;
#92015=DIRECTION ( 'NONE',  ( 0.000000000000000000, 1.000000000000000000, 0.000000000000000000 ) ) ;
#92016=CARTESIAN_POINT ( 'NONE',  ( -10.85000000000000142, 2.500000000000000000, 2.265063509461097357 ) ) ;
#92018=CIRCLE ( 'NONE', #85658, 0.1000000000000000472 ) ;
#92019=DIRECTION ( 'NONE',  ( 0.000000000000000000, 0.000000000000000000, 1.000000000000000000 ) ) ;
#92020=DIRECTION ( 'NONE',  ( -4.274815082592931898E-19, -0.9999939076577903929, -0.003490651415223739937 ) ) ;
#92021=DIRECTION ( 'NONE',  ( -0.000000000000000000, -1.000000000000000000, -0.000000000000000000 ) ) ;
#92022=VECTOR ( 'NONE', #90937, 1000.000000000000000 ) ;
#92023=EDGE_LOOP ( 'NONE', ( #23765, #13819, #41983, #7206 ) ) ;
#92024=CIRCLE ( 'NONE', #18857, 0.1000000000000002554 ) ;
#92026=PLANE ( 'NONE',  #5679 ) ;
#92027=DIRECTION ( 'NONE',  ( -0.000000000000000000, 1.000000000000000000, -0.000000000000000000 ) ) ;
#92028=DIRECTION ( 'NONE',  ( 0.000000000000000000, 1.000000000000000000, 0.000000000000000000 ) ) ;
#92029=EDGE_LOOP ( 'NONE', ( #69637, #56916 ) ) ;
#92030=FACE_OUTER_BOUND ( 'NONE', #106848, .T. ) ;
#92031=ADVANCED_FACE ( 'NONE', ( #77844 ), #127771, .T. ) ;
#92032=CARTESIAN_POINT ( 'NONE',  ( 13.09999999999990195, 12.50000000000000000, -3.918623584224389056 ) ) ;
#92033=DIRECTION ( 'NONE',  ( -0.000000000000000000, 1.000000000000000000, -0.000000000000000000 ) ) ;
#92034=ORIENTED_EDGE ( 'NONE', *, *, #42138, .T. ) ;
#92035=ORIENTED_EDGE ( 'NONE', *, *, #94195, .T. ) ;
#92036=CARTESIAN_POINT ( 'NONE',  ( 3.749999999999938716, 12.50000000000000000, 7.188010851410848723 ) ) ;
#92037=EDGE_CURVE ( 'NONE', #93758, #10983, #7164, .T. ) ;
#92038=ORIENTED_EDGE ( 'NONE', *, *, #16740, .F. ) ;
#92039=VERTEX_POINT ( 'NONE', #48396 ) ;
#92040=DIRECTION ( 'NONE',  ( 0.000000000000000000, -0.000000000000000000, 1.000000000000000000 ) ) ;
#92041=CONICAL_SURFACE ( 'NONE', #106699, 0.1000000000000002554, 0.003490658503988666988 ) ;
#92042=AXIS2_PLACEMENT_3D ( 'NONE', #41776, #93433, #92800 ) ;
#92043=CARTESIAN_POINT ( 'NONE',  ( 20.69433222468020972, 2.585316282069821892, -4.139109617385188677 ) ) ;
#92045=DIRECTION ( 'NONE',  ( -0.000000000000000000, -1.000000000000000000, -0.000000000000000000 ) ) ;
#92046=VERTEX_POINT ( 'NONE', #28113 ) ;
#92047=AXIS2_PLACEMENT_3D ( 'NONE', #44762, #84671, #93218 ) ;
#92048=CARTESIAN_POINT ( 'NONE',  ( -3.350000000000032507, 12.50000000000000000, -6.495190528383302464 ) ) ;
#92049=ORIENTED_EDGE ( 'NONE', *, *, #117782, .T. ) ;
#92051=CARTESIAN_POINT ( 'NONE',  ( 12.69999999999989981, 2.500000000000000000, -0.2464101615137783419 ) ) ;
#92052=ORIENTED_EDGE ( 'NONE', *, *, #43197, .F. ) ;
#92053=VERTEX_POINT ( 'NONE', #78525 ) ;
#92054=ORIENTED_EDGE ( 'NONE', *, *, #95178, .T. ) ;
#92055=ORIENTED_EDGE ( 'NONE', *, *, #60683, .T. ) ;
#92056=DIRECTION ( 'NONE',  ( 0.000000000000000000, 0.000000000000000000, 1.000000000000000000 ) ) ;
#92057=CARTESIAN_POINT ( 'NONE',  ( 16.56576425165006583, 1.499999999999999334, 6.084390597445812787 ) ) ;
#92058=CARTESIAN_POINT ( 'NONE',  ( 4.399999999999940847, 12.50000000000000000, -3.983716857408426293 ) ) ;
#92059=FACE_BOUND ( 'NONE', #56552, .T. ) ;
#92060=VERTEX_POINT ( 'NONE', #27446 ) ;
#92062=FACE_OUTER_BOUND ( 'NONE', #45313, .T. ) ;
#92064=EDGE_CURVE ( 'NONE', #105417, #87541, #117275, .T. ) ;
#92065=DIRECTION ( 'NONE',  ( -0.000000000000000000, -1.000000000000000000, -0.000000000000000000 ) ) ;
#92066=CARTESIAN_POINT ( 'NONE',  ( -9.550000000000006040, 2.500000000000000000, -2.165063509461101710 ) ) ;
#92067=FACE_OUTER_BOUND ( 'NONE', #42150, .T. ) ;
#92068=VECTOR ( 'NONE', #7319, 1000.000000000000000 ) ;
#92069=EDGE_CURVE ( 'NONE', #30053, #94650, #46449, .T. ) ;
#92070=AXIS2_PLACEMENT_3D ( 'NONE', #94722, #63982, #103909 ) ;
#92071=FACE_OUTER_BOUND ( 'NONE', #118520, .T. ) ;
#92072=ORIENTED_EDGE ( 'NONE', *, *, #100378, .T. ) ;
#92073=VERTEX_POINT ( 'NONE', #107960 ) ;
#92074=ORIENTED_EDGE ( 'NONE', *, *, #55143, .T. ) ;
#92075=ORIENTED_EDGE ( 'NONE', *, *, #11089, .F. ) ;
#92076=EDGE_LOOP ( 'NONE', ( #52284, #104723, #21483, #102281 ) ) ;
#92079=FACE_OUTER_BOUND ( 'NONE', #108477, .T. ) ;
#92080=VERTEX_POINT ( 'NONE', #126960 ) ;
#92081=FACE_BOUND ( 'NONE', #118103, .T. ) ;
#92082=EDGE_CURVE ( 'NONE', #32290, #126580, #66734, .T. ) ;
#92083=AXIS2_PLACEMENT_3D ( 'NONE', #3672, #24609, #33773 ) ;
#92085=EDGE_CURVE ( 'NONE', #19127, #82397, #104761, .T. ) ;
#92086=ORIENTED_EDGE ( 'NONE', *, *, #22881, .F. ) ;
#92087=CARTESIAN_POINT ( 'NONE',  ( -3.750000000000031086, 2.500000000000000000, -5.802370205355749988 ) ) ;
#92088=DIRECTION ( 'NONE',  ( -0.000000000000000000, 1.000000000000000000, -0.000000000000000000 ) ) ;
#92089=EDGE_CURVE ( 'NONE', #126865, #21052, #98130, .T. ) ;
#92090=DIRECTION ( 'NONE',  ( -0.000000000000000000, 1.000000000000000000, -0.000000000000000000 ) ) ;
#92091=VERTEX_POINT ( 'NONE', #88295 ) ;
#92092=CARTESIAN_POINT ( 'NONE',  ( -4.600000000000028066, 2.500000000000000000, -3.737306695894649700 ) ) ;
#92093=VECTOR ( 'NONE', #34751, 1000.000000000000000 ) ;
#92094=ORIENTED_EDGE ( 'NONE', *, *, #62405, .F. ) ;
#92095=AXIS2_PLACEMENT_3D ( 'NONE', #121673, #22862, #89800 ) ;
#92097=EDGE_LOOP ( 'NONE', ( #120875, #43039, #110344, #68160 ) ) ;
#92098=EDGE_LOOP ( 'NONE', ( #67617, #74875 ) ) ;
#92099=DIRECTION ( 'NONE',  ( 0.000000000000000000, 0.000000000000000000, -1.000000000000000000 ) ) ;
#92100=CARTESIAN_POINT ( 'NONE',  ( 11.24999999999990585, 2.500000000000000000, -5.802370205355749988 ) ) ;
#92101=ORIENTED_EDGE ( 'NONE', *, *, #105703, .T. ) ;
#92102=LINE ( 'NONE', #112407, #62194 ) ;
#92103=AXIS2_PLACEMENT_3D ( 'NONE', #107189, #105917, #35885 ) ;
#92104=DIRECTION ( 'NONE',  ( -0.000000000000000000, -1.000000000000000000, -0.000000000000000000 ) ) ;
#92105=CARTESIAN_POINT ( 'NONE',  ( -1.650000000000035216, 12.50000000000000000, -1.407149913249512663 ) ) ;
#92106=CARTESIAN_POINT ( 'NONE',  ( 0.1999999999999636513, 2.500000000000000000, -0.4464101615137760493 ) ) ;
#92107=CIRCLE ( 'NONE', #39906, 0.09999999999999982514 ) ;
#92108=CARTESIAN_POINT ( 'NONE',  ( 10.64999999999991331, 12.50000000000000000, -2.511473670974877948 ) ) ;
#92109=VERTEX_POINT ( 'NONE', #28767 ) ;
#92110=CARTESIAN_POINT ( 'NONE',  ( 2.499999999999947153, 2.500000000000000000, -3.737306695894649700 ) ) ;
#92111=ORIENTED_EDGE ( 'NONE', *, *, #9037, .T. ) ;
#92112=DIRECTION ( 'NONE',  ( 0.000000000000000000, 0.000000000000000000, 1.000000000000000000 ) ) ;
#92113=ORIENTED_EDGE ( 'NONE', *, *, #26378, .T. ) ;
#92114=FACE_OUTER_BOUND ( 'NONE', #32067, .T. ) ;
#92115=ORIENTED_EDGE ( 'NONE', *, *, #34968, .F. ) ;
#92116=DIRECTION ( 'NONE',  ( -0.000000000000000000, -1.000000000000000000, -0.000000000000000000 ) ) ;
#92117=CARTESIAN_POINT ( 'NONE',  ( -10.84999999999999964, 12.50000000000000000, 2.792790559304612064 ) ) ;
#92118=CARTESIAN_POINT ( 'NONE',  ( 12.09999999999990550, 2.500000000000000000, -4.330127018922201643 ) ) ;
#92120=FACE_OUTER_BOUND ( 'NONE', #70627, .T. ) ;
#92121=VERTEX_POINT ( 'NONE', #37930 ) ;
#92122=ORIENTED_EDGE ( 'NONE', *, *, #26645, .F. ) ;
#92125=AXIS2_PLACEMENT_3D ( 'NONE', #88440, #83158, #14382 ) ;
#92126=DIRECTION ( 'NONE',  ( 0.000000000000000000, -0.000000000000000000, 1.000000000000000000 ) ) ;
#92127=EDGE_CURVE ( 'NONE', #57128, #121644, #121491, .T. ) ;
#92128=VERTEX_POINT ( 'NONE', #49058 ) ;
#92129=ORIENTED_EDGE ( 'NONE', *, *, #113289, .T. ) ;
#92130=ORIENTED_EDGE ( 'NONE', *, *, #101497, .T. ) ;
#92131=CIRCLE ( 'NONE', #23176, 0.1000000000000002554 ) ;
#92132=EDGE_CURVE ( 'NONE', #5978, #37903, #88968, .T. ) ;
#92133=AXIS2_PLACEMENT_3D ( 'NONE', #17425, #37099, #116918 ) ;
#92134=DIRECTION ( 'NONE',  ( 0.000000000000000000, 1.000000000000000000, 0.000000000000000000 ) ) ;
#92135=ADVANCED_FACE ( 'NONE', ( #31993 ), #1224, .T. ) ;
#92136=ADVANCED_FACE ( 'NONE', ( #59535 ), #219, .T. ) ;
#92137=VERTEX_POINT ( 'NONE', #19580 ) ;
#92138=CARTESIAN_POINT ( 'NONE',  ( -12.29999999999999361, 2.500000000000000000, 3.983716857408420076 ) ) ;
#92139=LINE ( 'NONE', #90859, #95848 ) ;
#92140=AXIS2_PLACEMENT_3D ( 'NONE', #75448, #127151, #35550 ) ;
#92141=CARTESIAN_POINT ( 'NONE',  ( -7.900000000000014566, 2.500000000000000000, -4.330127018922201643 ) ) ;
#92142=ORIENTED_EDGE ( 'NONE', *, *, #129092, .T. ) ;
#92143=DIRECTION ( 'NONE',  ( 0.000000000000000000, 0.000000000000000000, -1.000000000000000000 ) ) ;
#92144=DIRECTION ( 'NONE',  ( 0.000000000000000000, 0.000000000000000000, -1.000000000000000000 ) ) ;
#92145=EDGE_CURVE ( 'NONE', #108759, #129486, #18994, .T. ) ;
#92146=CARTESIAN_POINT ( 'NONE',  ( 11.24999999999990763, 2.500000000000000000, 1.472243186433545459 ) ) ;
#92147=DIRECTION ( 'NONE',  ( 0.000000000000000000, -0.9999939076577903929, 0.003490651415223739937 ) ) ;
#92148=AXIS2_PLACEMENT_3D ( 'NONE', #72984, #100502, #72355 ) ;
#92149=CARTESIAN_POINT ( 'NONE',  ( -13.74999999999998757, 12.50000000000000000, -2.792790559304614284 ) ) ;
#92150=ORIENTED_EDGE ( 'NONE', *, *, #124593, .F. ) ;
#92151=ADVANCED_FACE ( 'NONE', ( #9758 ), #56644, .T. ) ;
#92152=CARTESIAN_POINT ( 'NONE',  ( -6.850000000000017408, 12.50000000000000000, -6.148780366869526226 ) ) ;
#92153=EDGE_CURVE ( 'NONE', #94042, #86969, #2494, .T. ) ;
#92154=CARTESIAN_POINT ( 'NONE',  ( 21.23528140090950700, -2.699413673072311504, 2.293764360948885805 ) ) ;
#92156=VERTEX_POINT ( 'NONE', #71247 ) ;
#92158=DIRECTION ( 'NONE',  ( 0.000000000000000000, 0.000000000000000000, -1.000000000000000000 ) ) ;
#92159=DIRECTION ( 'NONE',  ( 0.000000000000000000, 0.000000000000000000, -1.000000000000000000 ) ) ;
#92160=EDGE_CURVE ( 'NONE', #41592, #71750, #2277, .T. ) ;
#92161=CARTESIAN_POINT ( 'NONE',  ( -2.300000000000032685, 2.500000000000000000, -4.576537180435978236 ) ) ;
#92162=DIRECTION ( 'NONE',  ( -0.000000000000000000, 1.000000000000000000, -0.000000000000000000 ) ) ;
#92163=AXIS2_PLACEMENT_3D ( 'NONE', #34010, #24193, #93577 ) ;
#92164=DIRECTION ( 'NONE',  ( 0.000000000000000000, 0.000000000000000000, 1.000000000000000000 ) ) ;
#92165=CARTESIAN_POINT ( 'NONE',  ( -6.850000000000013856, 2.500000000000000000, 1.918653347947321564 ) ) ;
#92166=DIRECTION ( 'NONE',  ( 0.000000000000000000, -0.000000000000000000, 1.000000000000000000 ) ) ;
#92167=LINE ( 'NONE', #80435, #50153 ) ;
#92168=AXIS2_PLACEMENT_3D ( 'NONE', #121001, #40533, #110533 ) ;
#92169=ORIENTED_EDGE ( 'NONE', *, *, #28576, .F. ) ;
#92170=AXIS2_PLACEMENT_3D ( 'NONE', #4239, #4884, #81536 ) ;
#92171=VERTEX_POINT ( 'NONE', #111833 ) ;
#92172=ORIENTED_EDGE ( 'NONE', *, *, #124899, .F. ) ;
#92173=ORIENTED_EDGE ( 'NONE', *, *, #24132, .F. ) ;
#92174=DIRECTION ( 'NONE',  ( 0.000000000000000000, 1.000000000000000000, 0.000000000000000000 ) ) ;
#92175=DIRECTION ( 'NONE',  ( -0.000000000000000000, -1.000000000000000000, -0.000000000000000000 ) ) ;
#92176=CONICAL_SURFACE ( 'NONE', #85908, 0.1000000000000002554, 0.003490658503988666988 ) ;
#92177=CIRCLE ( 'NONE', #54519, 0.06509327318403745899 ) ;
#92178=VERTEX_POINT ( 'NONE', #22181 ) ;
#92179=PLANE ( 'NONE',  #125953 ) ;
#92180=CARTESIAN_POINT ( 'NONE',  ( 11.89999999999990443, 12.50000000000000000, 0.3464101615137736845 ) ) ;
#92181=DIRECTION ( 'NONE',  ( -0.000000000000000000, 1.000000000000000000, -0.000000000000000000 ) ) ;
#92182=VERTEX_POINT ( 'NONE', #60167 ) ;
#92183=DIRECTION ( 'NONE',  ( -4.274815082592931898E-19, -0.9999939076577903929, -0.003490651415223739937 ) ) ;
#92184=DIRECTION ( 'NONE',  ( 0.000000000000000000, 0.000000000000000000, 1.000000000000000000 ) ) ;
#92185=AXIS2_PLACEMENT_3D ( 'NONE', #126823, #34600, #64036 ) ;
#92186=ORIENTED_EDGE ( 'NONE', *, *, #54244, .F. ) ;
#92187=VECTOR ( 'NONE', #57460, 1000.000000000000000 ) ;
#92188=EDGE_CURVE ( 'NONE', #121009, #29184, #35743, .T. ) ;
#92189=ORIENTED_EDGE ( 'NONE', *, *, #30089, .F. ) ;
#92190=ORIENTED_EDGE ( 'NONE', *, *, #76923, .F. ) ;
#92191=VERTEX_POINT ( 'NONE', #20227 ) ;
#92192=CARTESIAN_POINT ( 'NONE',  ( 10.19999999999991047, 2.500000000000000000, 4.576537180435972019 ) ) ;
#92193=AXIS2_PLACEMENT_3D ( 'NONE', #3685, #51511, #73075 ) ;
#92194=DIRECTION ( 'NONE',  ( 0.000000000000000000, -0.9999939076577903929, 0.003490651415223739937 ) ) ;
#92195=DIRECTION ( 'NONE',  ( -0.000000000000000000, -1.000000000000000000, -0.000000000000000000 ) ) ;
#92196=CARTESIAN_POINT ( 'NONE',  ( 3.549999999999941203, 12.50000000000000000, 6.213873640053559022 ) ) ;
#92197=ORIENTED_EDGE ( 'NONE', *, *, #97909, .F. ) ;
#92198=CIRCLE ( 'NONE', #46235, 0.1000000000000002554 ) ;
#92199=AXIS2_PLACEMENT_3D ( 'NONE', #22792, #73163, #24706 ) ;
#92200=CARTESIAN_POINT ( 'NONE',  ( -11.44999999999999751, 12.50000000000000000, 1.883746621131358934 ) ) ;
#92201=VERTEX_POINT ( 'NONE', #31349 ) ;
#92202=CARTESIAN_POINT ( 'NONE',  ( 10.59999999999990905, 2.500000000000000000, -3.883716857408426648 ) ) ;
#92203=DIRECTION ( 'NONE',  ( 0.000000000000000000, 0.000000000000000000, -1.000000000000000000 ) ) ;
#92204=CARTESIAN_POINT ( 'NONE',  ( 4.149999999999941735, 2.500000000000000000, -5.702370205355749455 ) ) ;
#92205=CARTESIAN_POINT ( 'NONE',  ( -4.800000000000024691, 2.500000000000000000, 0.3464101615137735735 ) ) ;
#92207=VERTEX_POINT ( 'NONE', #91543 ) ;
#92208=ORIENTED_EDGE ( 'NONE', *, *, #64941, .F. ) ;
#92209=CARTESIAN_POINT ( 'NONE',  ( 8.349999999999919709, 12.50000000000000000, -2.230156782645139391 ) ) ;
#92210=LINE ( 'NONE', #122980, #8011 ) ;
#92211=CARTESIAN_POINT ( 'NONE',  ( 2.699999999999946443, 2.500000000000000000, 0.4464101615137735513 ) ) ;
#92212=FACE_BOUND ( 'NONE', #108192, .T. ) ;
#92213=DIRECTION ( 'NONE',  ( -0.000000000000000000, -1.000000000000000000, -0.000000000000000000 ) ) ;
#92214=DIRECTION ( 'NONE',  ( -0.000000000000000000, 1.000000000000000000, -0.000000000000000000 ) ) ;
#92215=DIRECTION ( 'NONE',  ( 0.000000000000000000, 1.000000000000000000, 0.000000000000000000 ) ) ;
#92216=CIRCLE ( 'NONE', #75490, 0.09999999999999999167 ) ;
#92217=CIRCLE ( 'NONE', #35802, 0.06509327318403745899 ) ;
#92218=DIRECTION ( 'NONE',  ( 0.000000000000000000, -0.9999939076577903929, 0.003490651415223739937 ) ) ;
#92219=CONICAL_SURFACE ( 'NONE', #4464, 0.1000000000000000472, 0.003490658503988666988 ) ;
#92221=FACE_OUTER_BOUND ( 'NONE', #76713, .T. ) ;
#92222=VERTEX_POINT ( 'NONE', #20871 ) ;
#92223=CARTESIAN_POINT ( 'NONE',  ( 11.24999999999994316, 2.500000000000000000, -6.595190528383302109 ) ) ;
#92224=EDGE_CURVE ( 'NONE', #2627, #106863, #52456, .T. ) ;
#92225=CIRCLE ( 'NONE', #56705, 0.1000000000000002554 ) ;
#92226=DIRECTION ( 'NONE',  ( 0.000000000000000000, 1.000000000000000000, 0.000000000000000000 ) ) ;
#92227=AXIS2_PLACEMENT_3D ( 'NONE', #15481, #5656, #16114 ) ;
#92228=EDGE_LOOP ( 'NONE', ( #58720, #98987 ) ) ;
#92229=ORIENTED_EDGE ( 'NONE', *, *, #97919, .T. ) ;
#92230=AXIS2_PLACEMENT_3D ( 'NONE', #84733, #65731, #25161 ) ;
#92231=DIRECTION ( 'NONE',  ( 0.000000000000000000, 1.000000000000000000, 0.000000000000000000 ) ) ;
#92232=EDGE_CURVE ( 'NONE', #14173, #24264, #102008, .T. ) ;
#92233=CARTESIAN_POINT ( 'NONE',  ( -11.24999999999999822, 2.500000000000000000, 5.902370205355745192 ) ) ;
#92234=FACE_BOUND ( 'NONE', #75893, .T. ) ;
#92235=EDGE_CURVE ( 'NONE', #10651, #41348, #82383, .T. ) ;
#92236=CARTESIAN_POINT ( 'NONE',  ( 10.39999999999991154, 2.500000000000000000, -5.022947341949754119 ) ) ;
#92237=ADVANCED_FACE ( 'NONE', ( #52266 ), #50330, .T. ) ;
#92238=ADVANCED_FACE ( 'NONE', ( #30713 ), #4492, .T. ) ;
#92239=ORIENTED_EDGE ( 'NONE', *, *, #118613, .F. ) ;
#92240=LINE ( 'NONE', #79849, #36180 ) ;
#92241=ADVANCED_FACE ( 'NONE', ( #11030 ), #50990, .T. ) ;
#92242=EDGE_CURVE ( 'NONE', #46755, #4130, #2454, .T. ) ;
#92243=CARTESIAN_POINT ( 'NONE',  ( -13.74999999999998934, 12.50000000000000000, 2.922977105672690534 ) ) ;
#92245=ORIENTED_EDGE ( 'NONE', *, *, #48531, .T. ) ;
#92246=CARTESIAN_POINT ( 'NONE',  ( 12.29999999999990123, 2.500000000000000000, 0.3464101615137735735 ) ) ;
#92247=FACE_OUTER_BOUND ( 'NONE', #100425, .T. ) ;
#92248=ORIENTED_EDGE ( 'NONE', *, *, #90622, .T. ) ;
#92249=CARTESIAN_POINT ( 'NONE',  ( -3.150000000000033218, 2.500000000000000000, -6.741600689897078169 ) ) ;
#92250=PLANE ( 'NONE',  #65648 ) ;
#92251=ADVANCED_FACE ( 'NONE', ( #95411 ), #35837, .T. ) ;
#92252=CIRCLE ( 'NONE', #71412, 0.06509327318403741736 ) ;
#92253=AXIS2_PLACEMENT_3D ( 'NONE', #18591, #8748, #8117 ) ;
#92254=ORIENTED_EDGE ( 'NONE', *, *, #104752, .F. ) ;
#92255=DIRECTION ( 'NONE',  ( 0.000000000000000000, 0.000000000000000000, -1.000000000000000000 ) ) ;
#92256=LINE ( 'NONE', #42548, #99980 ) ;
#92257=DIRECTION ( 'NONE',  ( 0.000000000000000000, 0.000000000000000000, -1.000000000000000000 ) ) ;
#92258=ORIENTED_EDGE ( 'NONE', *, *, #35927, .F. ) ;
#92259=ORIENTED_EDGE ( 'NONE', *, *, #6252, .T. ) ;
#92260=FACE_OUTER_BOUND ( 'NONE', #1232, .T. ) ;
#92261=CIRCLE ( 'NONE', #81884, 0.09999999999999982514 ) ;
#92262=EDGE_LOOP ( 'NONE', ( #113274, #60073 ) ) ;
#92263=DIRECTION ( 'NONE',  ( 0.000000000000000000, 0.000000000000000000, 1.000000000000000000 ) ) ;
#92264=AXIS2_PLACEMENT_3D ( 'NONE', #124369, #126946, #34718 ) ;
#92265=DIRECTION ( 'NONE',  ( -0.000000000000000000, -1.000000000000000000, -0.000000000000000000 ) ) ;
#92266=PLANE ( 'NONE',  #46678 ) ;
#92267=ORIENTED_EDGE ( 'NONE', *, *, #129566, .F. ) ;
#92268=DIRECTION ( 'NONE',  ( -4.274815082592931898E-19, -0.9999939076577903929, -0.003490651415223739937 ) ) ;
#92269=DIRECTION ( 'NONE',  ( 0.000000000000000000, 0.000000000000000000, -1.000000000000000000 ) ) ;
#92270=DIRECTION ( 'NONE',  ( 0.000000000000000000, 0.000000000000000000, 1.000000000000000000 ) ) ;
#92271=DIRECTION ( 'NONE',  ( 0.000000000000000000, 0.000000000000000000, 1.000000000000000000 ) ) ;
#92272=DIRECTION ( 'NONE',  ( 0.000000000000000000, 0.000000000000000000, -1.000000000000000000 ) ) ;
#92273=DIRECTION ( 'NONE',  ( 0.000000000000000000, 0.000000000000000000, 1.000000000000000000 ) ) ;
#92274=VECTOR ( 'NONE', #91401, 1000.000000000000000 ) ;
#92275=EDGE_LOOP ( 'NONE', ( #15599, #85410 ) ) ;
#92277=AXIS2_PLACEMENT_3D ( 'NONE', #112198, #287, #50695 ) ;
#92278=EDGE_LOOP ( 'NONE', ( #45728, #101736, #56313, #70970 ) ) ;
#92279=DIRECTION ( 'NONE',  ( 0.000000000000000000, 0.000000000000000000, -1.000000000000000000 ) ) ;
#92280=EDGE_LOOP ( 'NONE', ( #86962, #30100, #54931, #34294 ) ) ;
#92281=DIRECTION ( 'NONE',  ( 0.000000000000000000, 0.000000000000000000, 1.000000000000000000 ) ) ;
#92282=VECTOR ( 'NONE', #114887, 1000.000000000000000 ) ;
#92283=ADVANCED_FACE ( 'NONE', ( #112480 ), #22821, .T. ) ;
#92284=ORIENTED_EDGE ( 'NONE', *, *, #4771, .T. ) ;
#92285=EDGE_LOOP ( 'NONE', ( #55692, #40898, #94039, #57645 ) ) ;
#92286=EDGE_LOOP ( 'NONE', ( #86662, #17006, #126472, #111320 ) ) ;
#92287=ADVANCED_FACE ( 'NONE', ( #52912 ), #100659, .T. ) ;
#92288=DIRECTION ( 'NONE',  ( 0.000000000000000000, -0.9999939076577903929, 0.003490651415223739937 ) ) ;
#92289=CONICAL_SURFACE ( 'NONE', #127898, 0.1000000000000000472, 0.003490658503988666988 ) ;
#92290=EDGE_CURVE ( 'NONE', #79082, #76513, #27489, .T. ) ;
#92291=DIRECTION ( 'NONE',  ( 0.000000000000000000, -0.000000000000000000, 1.000000000000000000 ) ) ;
#92292=DIRECTION ( 'NONE',  ( -0.000000000000000000, 1.000000000000000000, -0.000000000000000000 ) ) ;
#92293=EDGE_CURVE ( 'NONE', #54837, #98287, #37977, .T. ) ;
#92294=CARTESIAN_POINT ( 'NONE',  ( 12.29999999999990479, 2.500000000000000000, 4.776537180435972196 ) ) ;
#92295=AXIS2_PLACEMENT_3D ( 'NONE', #129151, #107551, #68904 ) ;
#92296=VECTOR ( 'NONE', #3618, 1000.000000000000000 ) ;
#92297=PLANE ( 'NONE',  #29225 ) ;
#92298=DIRECTION ( 'NONE',  ( 0.000000000000000000, -0.000000000000000000, 1.000000000000000000 ) ) ;
#92299=DIRECTION ( 'NONE',  ( -0.000000000000000000, -1.000000000000000000, -0.000000000000000000 ) ) ;
#92300=FACE_OUTER_BOUND ( 'NONE', #42155, .T. ) ;
#92301=ADVANCED_FACE ( 'NONE', ( #93481 ), #54201, .T. ) ;
#92302=DIRECTION ( 'NONE',  ( 0.000000000000000000, -0.000000000000000000, 1.000000000000000000 ) ) ;
#92303=ADVANCED_FACE ( 'NONE', ( #122305 ), #56729, .T. ) ;
#92304=EDGE_CURVE ( 'NONE', #75397, #82798, #31724, .T. ) ;
#92305=ORIENTED_EDGE ( 'NONE', *, *, #69098, .T. ) ;
#92306=EDGE_CURVE ( 'NONE', #3120, #31226, #302, .T. ) ;
#92307=DIRECTION ( 'NONE',  ( 0.000000000000000000, 1.000000000000000000, 0.000000000000000000 ) ) ;
#92308=ORIENTED_EDGE ( 'NONE', *, *, #43261, .T. ) ;
#92309=EDGE_LOOP ( 'NONE', ( #52967, #29756 ) ) ;
#92310=DIRECTION ( 'NONE',  ( -0.000000000000000000, -1.000000000000000000, -0.000000000000000000 ) ) ;
#92311=CARTESIAN_POINT ( 'NONE',  ( 0.3999999999999563904, 12.50000000000000000, 3.637306695894644726 ) ) ;
#92312=DIRECTION ( 'NONE',  ( 0.000000000000000000, 1.000000000000000000, 0.000000000000000000 ) ) ;
#92313=ADVANCED_FACE ( 'NONE', ( #23439 ), #104863, .T. ) ;
#92315=DIRECTION ( 'NONE',  ( 0.000000000000000000, 0.000000000000000000, -1.000000000000000000 ) ) ;
#92316=AXIS2_PLACEMENT_3D ( 'NONE', #120412, #21563, #60842 ) ;
#92317=DIRECTION ( 'NONE',  ( 0.000000000000000000, 1.000000000000000000, 0.000000000000000000 ) ) ;
#92318=ORIENTED_EDGE ( 'NONE', *, *, #41938, .T. ) ;
#92319=CIRCLE ( 'NONE', #8672, 0.06509327318403745899 ) ;
#92320=AXIS2_PLACEMENT_3D ( 'NONE', #57048, #7955, #126460 ) ;
#92321=ORIENTED_EDGE ( 'NONE', *, *, #119744, .T. ) ;
#92322=VECTOR ( 'NONE', #7030, 1000.000000000000000 ) ;
#92323=ORIENTED_EDGE ( 'NONE', *, *, #9624, .T. ) ;
#92324=CONICAL_SURFACE ( 'NONE', #2425, 0.1000000000000000472, 0.003490658503988666988 ) ;
#92325=ORIENTED_EDGE ( 'NONE', *, *, #54390, .T. ) ;
#92326=CIRCLE ( 'NONE', #121567, 0.09999999999999999167 ) ;
#92327=EDGE_CURVE ( 'NONE', #98142, #48660, #92252, .T. ) ;
#92328=ORIENTED_EDGE ( 'NONE', *, *, #4470, .T. ) ;
#92329=FACE_OUTER_BOUND ( 'NONE', #80253, .T. ) ;
#92330=DIRECTION ( 'NONE',  ( 0.000000000000000000, -0.9999939076577903929, 0.003490651415223739937 ) ) ;
#92331=DIRECTION ( 'NONE',  ( 0.000000000000000000, 0.000000000000000000, 1.000000000000000000 ) ) ;
#92332=DIRECTION ( 'NONE',  ( -0.000000000000000000, -1.000000000000000000, -0.000000000000000000 ) ) ;
#92333=CARTESIAN_POINT ( 'NONE',  ( -9.999999999999969802, 2.500000000000000000, 4.430127018922196847 ) ) ;
#92334=EDGE_LOOP ( 'NONE', ( #112890, #35528 ) ) ;
#92335=DIRECTION ( 'NONE',  ( -0.000000000000000000, 1.000000000000000000, -0.000000000000000000 ) ) ;
#92336=DIRECTION ( 'NONE',  ( 0.000000000000000000, 0.000000000000000000, -1.000000000000000000 ) ) ;
#92337=DIRECTION ( 'NONE',  ( 0.000000000000000000, 1.000000000000000000, 0.000000000000000000 ) ) ;
#92338=FACE_OUTER_BOUND ( 'NONE', #14132, .T. ) ;
#92339=ORIENTED_EDGE ( 'NONE', *, *, #19553, .T. ) ;
#92340=ADVANCED_FACE ( 'NONE', ( #35217 ), #125695, .T. ) ;
#92342=VERTEX_POINT ( 'NONE', #63375 ) ;
#92343=DIRECTION ( 'NONE',  ( -0.000000000000000000, -1.000000000000000000, -0.000000000000000000 ) ) ;
#92344=VERTEX_POINT ( 'NONE', #113768 ) ;
#92345=DIRECTION ( 'NONE',  ( 0.000000000000000000, 0.000000000000000000, 1.000000000000000000 ) ) ;
#92346=CIRCLE ( 'NONE', #4583, 0.1000000000000002554 ) ;
#92347=CARTESIAN_POINT ( 'NONE',  ( -6.850000000000013856, 12.50000000000000000, 1.818653347947321475 ) ) ;
#92348=AXIS2_PLACEMENT_3D ( 'NONE', #98932, #40021, #79930 ) ;
#92349=ORIENTED_EDGE ( 'NONE', *, *, #3585, .T. ) ;
#92351=DIRECTION ( 'NONE',  ( 0.000000000000000000, 0.000000000000000000, -1.000000000000000000 ) ) ;
#92352=EDGE_CURVE ( 'NONE', #34347, #65457, #121592, .T. ) ;
#92353=CARTESIAN_POINT ( 'NONE',  ( 5.399999999999934630, 12.50000000000000000, 0.6928203230275494784 ) ) ;
#92354=DIRECTION ( 'NONE',  ( 0.000000000000000000, -0.000000000000000000, 1.000000000000000000 ) ) ;
#92355=VECTOR ( 'NONE', #66613, 1000.000000000000000 ) ;
#92356=VECTOR ( 'NONE', #74284, 1000.000000000000000 ) ;
#92357=AXIS2_PLACEMENT_3D ( 'NONE', #69463, #128428, #99594 ) ;
#92358=CARTESIAN_POINT ( 'NONE',  ( -9.400000000000007461, 2.500000000000000000, 3.983716857408420076 ) ) ;
#92359=CONICAL_SURFACE ( 'NONE', #109070, 0.1000000000000000056, 0.003490658503988666988 ) ;
#92360=CIRCLE ( 'NONE', #75627, 0.06509327318403745899 ) ;
#92361=ORIENTED_EDGE ( 'NONE', *, *, #88900, .F. ) ;
#92362=ORIENTED_EDGE ( 'NONE', *, *, #61659, .F. ) ;
#92364=DIRECTION ( 'NONE',  ( 0.000000000000000000, 0.000000000000000000, -1.000000000000000000 ) ) ;
#92365=CARTESIAN_POINT ( 'NONE',  ( -9.150000000000005684, 2.500000000000000000, 6.595190528383296780 ) ) ;
#92366=CIRCLE ( 'NONE', #104884, 0.1000000000000002554 ) ;
#92367=AXIS2_PLACEMENT_3D ( 'NONE', #95140, #93213, #15255 ) ;
#92368=PLANE ( 'NONE',  #39682 ) ;
#92369=VERTEX_POINT ( 'NONE', #13610 ) ;
#92370=AXIS2_PLACEMENT_3D ( 'NONE', #15259, #87235, #15917 ) ;
#92371=VECTOR ( 'NONE', #124521, 1000.000000000000000 ) ;
#92372=AXIS2_PLACEMENT_3D ( 'NONE', #78933, #126068, #117513 ) ;
#92373=ORIENTED_EDGE ( 'NONE', *, *, #116646, .F. ) ;
#92374=FACE_OUTER_BOUND ( 'NONE', #98495, .T. ) ;
#92375=LINE ( 'NONE', #72113, #53016 ) ;
#92376=CONICAL_SURFACE ( 'NONE', #79866, 0.1000000000000000472, 0.003490658503988666988 ) ;
#92377=CARTESIAN_POINT ( 'NONE',  ( 11.04999999999990834, 12.50000000000000000, 1.818653347947321475 ) ) ;
#92378=CARTESIAN_POINT ( 'NONE',  ( 3.149999999999942624, 2.500000000000000000, 6.941600689897073018 ) ) ;
#92379=ORIENTED_EDGE ( 'NONE', *, *, #40232, .F. ) ;
#92380=CARTESIAN_POINT ( 'NONE',  ( 3.949999999999939782, 12.50000000000000000, 2.576566944158910744 ) ) ;
#92381=EDGE_CURVE ( 'NONE', #30567, #117617, #102709, .T. ) ;
#92382=DIRECTION ( 'NONE',  ( 0.000000000000000000, 0.000000000000000000, 1.000000000000000000 ) ) ;
#92383=VECTOR ( 'NONE', #13843, 1000.000000000000000 ) ;
#92384=ORIENTED_EDGE ( 'NONE', *, *, #56967, .T. ) ;
#92386=ORIENTED_EDGE ( 'NONE', *, *, #20023, .T. ) ;
#92387=CARTESIAN_POINT ( 'NONE',  ( 6.049999999999935874, 12.50000000000000000, -6.841600689897077814 ) ) ;
#92388=VERTEX_POINT ( 'NONE', #43117 ) ;
#92389=DIRECTION ( 'NONE',  ( 0.000000000000000000, 0.000000000000000000, 1.000000000000000000 ) ) ;
#92390=CARTESIAN_POINT ( 'NONE',  ( 2.499999999999983569, 2.500000000000000000, -2.276824562219559311E-15 ) ) ;
#92391=EDGE_CURVE ( 'NONE', #60385, #90590, #96456, .T. ) ;
#92392=VERTEX_POINT ( 'NONE', #15539 ) ;
#92393=EDGE_CURVE ( 'NONE', #114671, #5769, #119441, .T. ) ;
#92394=ORIENTED_EDGE ( 'NONE', *, *, #29784, .F. ) ;
#92395=ADVANCED_FACE ( 'NONE', ( #83662 ), #98596, .T. ) ;
#92396=EDGE_CURVE ( 'NONE', #80227, #117538, #21247, .T. ) ;
#92397=DIRECTION ( 'NONE',  ( -0.000000000000000000, 1.000000000000000000, -0.000000000000000000 ) ) ;
#92398=CARTESIAN_POINT ( 'NONE',  ( 6.049999999999930544, 12.50000000000000000, 2.446380397790835826 ) ) ;
#92399=DIRECTION ( 'NONE',  ( 0.000000000000000000, 0.000000000000000000, 1.000000000000000000 ) ) ;
#92402=CONICAL_SURFACE ( 'NONE', #56882, 0.1000000000000002554, 0.003490658503988666988 ) ;
#92403=FACE_OUTER_BOUND ( 'NONE', #54659, .T. ) ;
#92404=CARTESIAN_POINT ( 'NONE',  ( -2.500000000000030642, 12.50000000000000000, -5.022947341949754119 ) ) ;
#92405=AXIS2_PLACEMENT_3D ( 'NONE', #38124, #116035, #46657 ) ;
#92406=CONICAL_SURFACE ( 'NONE', #109119, 0.1000000000000002554, 0.003490658503988666988 ) ;
#92407=FACE_OUTER_BOUND ( 'NONE', #1012, .T. ) ;
#92408=CARTESIAN_POINT ( 'NONE',  ( 6.849999999999929479, 2.500000000000000000, -2.611473670974877592 ) ) ;
#92409=ADVANCED_FACE ( 'NONE', ( #96672 ), #78361, .T. ) ;
#92410=EDGE_CURVE ( 'NONE', #107267, #113689, #58915, .T. ) ;
#92411=EDGE_CURVE ( 'NONE', #64286, #27855, #111112, .T. ) ;
#92412=AXIS2_PLACEMENT_3D ( 'NONE', #96193, #6498, #77219 ) ;
#92413=ORIENTED_EDGE ( 'NONE', *, *, #92393, .F. ) ;
#92415=CARTESIAN_POINT ( 'NONE',  ( 8.149999999999920419, 12.50000000000000000, 6.148780366869520897 ) ) ;
#92416=ORIENTED_EDGE ( 'NONE', *, *, #74525, .F. ) ;
#92417=DIRECTION ( 'NONE',  ( 0.000000000000000000, 0.000000000000000000, 1.000000000000000000 ) ) ;
#92418=DIRECTION ( 'NONE',  ( 0.000000000000000000, 0.000000000000000000, 1.000000000000000000 ) ) ;
#92419=CIRCLE ( 'NONE', #40204, 0.09999999999999982514 ) ;
#92420=DIRECTION ( 'NONE',  ( -0.000000000000000000, 1.000000000000000000, -0.000000000000000000 ) ) ;
#92421=CIRCLE ( 'NONE', #23466, 0.09999999999999982514 ) ;
#92422=ORIENTED_EDGE ( 'NONE', *, *, #10561, .T. ) ;
#92423=ORIENTED_EDGE ( 'NONE', *, *, #54716, .F. ) ;
#92425=FACE_BOUND ( 'NONE', #21530, .T. ) ;
#92426=ORIENTED_EDGE ( 'NONE', *, *, #29071, .T. ) ;
#92427=CARTESIAN_POINT ( 'NONE',  ( 11.04999999999990656, 2.500000000000000000, -6.148780366869526226 ) ) ;
#92428=CARTESIAN_POINT ( 'NONE',  ( 18.09027855933886997, -2.526462839860863507, 2.685672775344717156 ) ) ;
#92429=VECTOR ( 'NONE', #75739, 1000.000000000000000 ) ;
#92430=LINE ( 'NONE', #32890, #65965 ) ;
#92431=CARTESIAN_POINT ( 'NONE',  ( 10.64999999999990976, 2.500000000000000000, 1.818653347947321475 ) ) ;
#92432=FACE_OUTER_BOUND ( 'NONE', #34748, .T. ) ;
#92433=DIRECTION ( 'NONE',  ( -0.000000000000000000, -1.000000000000000000, -0.000000000000000000 ) ) ;
#92434=CARTESIAN_POINT ( 'NONE',  ( -10.84999999999999964, 12.50000000000000000, 7.188010851410848723 ) ) ;
#92435=CARTESIAN_POINT ( 'NONE',  ( -11.84999999999999787, 12.50000000000000000, -6.841600689897074261 ) ) ;
#92436=CARTESIAN_POINT ( 'NONE',  ( 7.699999999999923794, 12.50000000000000000, -0.3464101615137783474 ) ) ;
#92437=CARTESIAN_POINT ( 'NONE',  ( -3.750000000000025757, 12.50000000000000000, -2.857883832488653741 ) ) ;
#92438=DIRECTION ( 'NONE',  ( -0.000000000000000000, 1.000000000000000000, -0.000000000000000000 ) ) ;
#92439=ORIENTED_EDGE ( 'NONE', *, *, #28433, .F. ) ;
#92440=ORIENTED_EDGE ( 'NONE', *, *, #97191, .T. ) ;
#92442=DIRECTION ( 'NONE',  ( -0.000000000000000000, 1.000000000000000000, -0.000000000000000000 ) ) ;
#92443=EDGE_LOOP ( 'NONE', ( #102818, #116392, #28687, #36876 ) ) ;
#92444=CARTESIAN_POINT ( 'NONE',  ( -1.250000000000037526, 12.50000000000000000, -5.802370205355749988 ) ) ;
#92445=CARTESIAN_POINT ( 'NONE',  ( -8.550000000000009592, 2.500000000000000000, 6.741600689897071952 ) ) ;
#92446=ORIENTED_EDGE ( 'NONE', *, *, #103233, .T. ) ;
#92447=ORIENTED_EDGE ( 'NONE', *, *, #10991, .T. ) ;
#92448=ORIENTED_EDGE ( 'NONE', *, *, #111341, .F. ) ;
#92449=CARTESIAN_POINT ( 'NONE',  ( -11.44999999999999751, 12.50000000000000000, 6.148780366869520897 ) ) ;
#92450=DIRECTION ( 'NONE',  ( 0.000000000000000000, 0.000000000000000000, -1.000000000000000000 ) ) ;
#92451=( LENGTH_UNIT ( ) NAMED_UNIT ( * ) SI_UNIT ( .MILLI., .METRE. ) );
#92452=DIRECTION ( 'NONE',  ( 0.000000000000000000, 0.000000000000000000, 1.000000000000000000 ) ) ;
#92453=DIRECTION ( 'NONE',  ( 0.000000000000000000, 1.000000000000000000, 0.000000000000000000 ) ) ;
#92454=PLANE ( 'NONE',  #78961 ) ;
#92455=ORIENTED_EDGE ( 'NONE', *, *, #6715, .F. ) ;
#92456=CONICAL_SURFACE ( 'NONE', #59013, 0.1000000000000002554, 0.003490658503988666988 ) ;
#92457=CIRCLE ( 'NONE', #27699, 0.1000000000000002554 ) ;
#92458=FACE_OUTER_BOUND ( 'NONE', #92023, .T. ) ;
#92460=ADVANCED_FACE ( 'NONE', ( #97977 ), #77682, .T. ) ;
#92461=AXIS2_PLACEMENT_3D ( 'NONE', #78772, #119967, #49318 ) ;
#92462=VERTEX_POINT ( 'NONE', #126806 ) ;
#92463=AXIS2_PLACEMENT_3D ( 'NONE', #28451, #125349, #77529 ) ;
#92464=ORIENTED_EDGE ( 'NONE', *, *, #1237, .T. ) ;
#92465=EDGE_CURVE ( 'NONE', #25375, #70406, #14954, .T. ) ;
#92466=ORIENTED_EDGE ( 'NONE', *, *, #104111, .F. ) ;
#92467=ORIENTED_EDGE ( 'NONE', *, *, #8777, .T. ) ;
#92468=ORIENTED_EDGE ( 'NONE', *, *, #12754, .F. ) ;
#92469=AXIS2_PLACEMENT_3D ( 'NONE', #77253, #97526, #47153 ) ;
#92470=CARTESIAN_POINT ( 'NONE',  ( 9.399999999999915090, 2.500000000000000000, 3.883716857408421319 ) ) ;
#92471=ADVANCED_FACE ( 'NONE', ( #87500 ), #75529, .T. ) ;
#92472=CIRCLE ( 'NONE', #6666, 0.06509327318403743123 ) ;
#92473=DIRECTION ( 'NONE',  ( 0.000000000000000000, 1.000000000000000000, 0.000000000000000000 ) ) ;
#92474=DIRECTION ( 'NONE',  ( 0.000000000000000000, 1.000000000000000000, 0.000000000000000000 ) ) ;
#92475=CIRCLE ( 'NONE', #121711, 0.1000000000000002554 ) ;
#92476=PLANE ( 'NONE',  #124368 ) ;
#92477=CONICAL_SURFACE ( 'NONE', #6765, 0.1000000000000000472, 0.003490658503988666988 ) ;
#92478=VECTOR ( 'NONE', #102893, 1000.000000000000000 ) ;
#92479=FACE_OUTER_BOUND ( 'NONE', #73345, .T. ) ;
#92480=DIRECTION ( 'NONE',  ( -0.000000000000000000, -1.000000000000000000, -0.000000000000000000 ) ) ;
#92481=ORIENTED_EDGE ( 'NONE', *, *, #17914, .F. ) ;
#92482=DIRECTION ( 'NONE',  ( 0.000000000000000000, 1.000000000000000000, 0.000000000000000000 ) ) ;
#92483=ORIENTED_EDGE ( 'NONE', *, *, #26685, .T. ) ;
#92484=AXIS2_PLACEMENT_3D ( 'NONE', #35291, #54274, #24813 ) ;
#92485=CARTESIAN_POINT ( 'NONE',  ( 5.599999999999934808, 2.500000000000000000, -4.776537180435978414 ) ) ;
#92486=ORIENTED_EDGE ( 'NONE', *, *, #98480, .T. ) ;
#92487=DIRECTION ( 'NONE',  ( -0.000000000000000000, -1.000000000000000000, -0.000000000000000000 ) ) ;
#92488=ORIENTED_EDGE ( 'NONE', *, *, #49759, .T. ) ;
#92489=DIRECTION ( 'NONE',  ( -0.000000000000000000, 1.000000000000000000, -0.000000000000000000 ) ) ;
#92490=DIRECTION ( 'NONE',  ( 0.000000000000000000, 0.000000000000000000, 1.000000000000000000 ) ) ;
#92491=ORIENTED_EDGE ( 'NONE', *, *, #65772, .T. ) ;
#92492=ORIENTED_EDGE ( 'NONE', *, *, #107516, .T. ) ;
#92493=CARTESIAN_POINT ( 'NONE',  ( 1.249999999999952038, 2.500000000000000000, 5.802370205355744659 ) ) ;
#92494=LINE ( 'NONE', #4106, #11764 ) ;
#92495=AXIS2_PLACEMENT_3D ( 'NONE', #114074, #104254, #4102 ) ;
#92496=FACE_OUTER_BOUND ( 'NONE', #48508, .T. ) ;
#92497=DIRECTION ( 'NONE',  ( 0.000000000000000000, 0.000000000000000000, 1.000000000000000000 ) ) ;
#92498=CARTESIAN_POINT ( 'NONE',  ( 3.549999999999941203, 12.50000000000000000, 6.083687093685483660 ) ) ;
#92499=ORIENTED_EDGE ( 'NONE', *, *, #67985, .F. ) ;
#92500=EDGE_CURVE ( 'NONE', #45029, #18481, #79747, .T. ) ;
#92501=FACE_OUTER_BOUND ( 'NONE', #58382, .T. ) ;
#92502=AXIS2_PLACEMENT_3D ( 'NONE', #14626, #4812, #23838 ) ;
#92503=AXIS2_PLACEMENT_3D ( 'NONE', #44468, #85029, #95504 ) ;
#92504=AXIS2_PLACEMENT_3D ( 'NONE', #93614, #112618, #43246 ) ;
#92505=ORIENTED_EDGE ( 'NONE', *, *, #99513, .F. ) ;
#92506=CARTESIAN_POINT ( 'NONE',  ( -3.100000000000028511, 2.500000000000000000, -4.083716857408426826 ) ) ;
#92507=DIRECTION ( 'NONE',  ( 0.000000000000000000, 1.000000000000000000, 0.000000000000000000 ) ) ;
#92508=AXIS2_PLACEMENT_3D ( 'NONE', #47741, #38582, #117736 ) ;
#92509=CONICAL_SURFACE ( 'NONE', #82150, 0.09999999999999982514, 0.003490658503988666988 ) ;
#92510=VECTOR ( 'NONE', #77159, 1000.000000000000000 ) ;
#92511=EDGE_CURVE ( 'NONE', #24530, #110285, #33770, .T. ) ;
#92512=VECTOR ( 'NONE', #47721, 1000.000000000000000 ) ;
#92514=DIRECTION ( 'NONE',  ( 0.000000000000000000, 0.000000000000000000, 1.000000000000000000 ) ) ;
#92515=DIRECTION ( 'NONE',  ( 0.000000000000000000, 0.000000000000000000, -1.000000000000000000 ) ) ;
#92516=ADVANCED_FACE ( 'NONE', ( #26672 ), #117451, .T. ) ;
#92517=DIRECTION ( 'NONE',  ( 0.000000000000000000, 0.000000000000000000, -1.000000000000000000 ) ) ;
#92518=DIRECTION ( 'NONE',  ( -0.000000000000000000, -1.000000000000000000, -0.000000000000000000 ) ) ;
#92519=ORIENTED_EDGE ( 'NONE', *, *, #48253, .T. ) ;
#92520=VECTOR ( 'NONE', #63202, 1000.000000000000000 ) ;
#92521=FACE_OUTER_BOUND ( 'NONE', #62328, .T. ) ;
#92522=CARTESIAN_POINT ( 'NONE',  ( 3.099999999999945022, 2.500000000000000000, -4.676537180435978769 ) ) ;
#92523=LINE ( 'NONE', #41523, #129180 ) ;
#92524=VERTEX_POINT ( 'NONE', #126156 ) ;
#92526=ORIENTED_EDGE ( 'NONE', *, *, #99074, .F. ) ;
#92527=DIRECTION ( 'NONE',  ( 0.000000000000000000, 0.000000000000000000, 1.000000000000000000 ) ) ;
#92528=ORIENTED_EDGE ( 'NONE', *, *, #13888, .F. ) ;
#92529=VERTEX_POINT ( 'NONE', #77057 ) ;
#92530=DIRECTION ( 'NONE',  ( 0.000000000000000000, 0.000000000000000000, 1.000000000000000000 ) ) ;
#92531=ORIENTED_EDGE ( 'NONE', *, *, #3279, .F. ) ;
#92532=CARTESIAN_POINT ( 'NONE',  ( 17.17539648375208472, -2.541523116373817892, -5.507477068185379743 ) ) ;
#92533=DIRECTION ( 'NONE',  ( 0.000000000000000000, -0.000000000000000000, 1.000000000000000000 ) ) ;
#92534=DIRECTION ( 'NONE',  ( -0.000000000000000000, 1.000000000000000000, -0.000000000000000000 ) ) ;
#92535=CIRCLE ( 'NONE', #90375, 0.1000000000000000472 ) ;
#92536=ORIENTED_EDGE ( 'NONE', *, *, #56503, .T. ) ;
#92537=AXIS2_PLACEMENT_3D ( 'NONE', #74372, #96570, #114292 ) ;
#92538=CIRCLE ( 'NONE', #117554, 0.06509327318403745899 ) ;
#92539=DIRECTION ( 'NONE',  ( 0.000000000000000000, 0.000000000000000000, 1.000000000000000000 ) ) ;
#92540=EDGE_CURVE ( 'NONE', #10375, #65577, #104947, .T. ) ;
#92541=CARTESIAN_POINT ( 'NONE',  ( 9.149999999999918643, 2.500000000000000000, 2.265063509461097357 ) ) ;
#92542=AXIS2_PLACEMENT_3D ( 'NONE', #53750, #3362, #101080 ) ;
#92543=ORIENTED_EDGE ( 'NONE', *, *, #126610, .F. ) ;
#92544=AXIS2_PLACEMENT_3D ( 'NONE', #73169, #82360, #3145 ) ;
#92545=CONICAL_SURFACE ( 'NONE', #94695, 0.09999999999999999167, 0.003490658503988666988 ) ;
#92546=EDGE_CURVE ( 'NONE', #72305, #81664, #73560, .T. ) ;
#92547=VECTOR ( 'NONE', #102804, 1000.000000000000000 ) ;
#92548=ORIENTED_EDGE ( 'NONE', *, *, #59953, .T. ) ;
#92549=VERTEX_POINT ( 'NONE', #8941 ) ;
#92550=DIRECTION ( 'NONE',  ( 0.000000000000000000, 0.000000000000000000, -1.000000000000000000 ) ) ;
#92551=CARTESIAN_POINT ( 'NONE',  ( -1.250000000000001554, 12.50000000000000000, 2.165063509461097713 ) ) ;
#92552=CARTESIAN_POINT ( 'NONE',  ( 1.899999999999951283, 2.500000000000000000, -0.3464101615137782364 ) ) ;
#92553=EDGE_CURVE ( 'NONE', #7138, #35674, #85584, .T. ) ;
#92554=EDGE_CURVE ( 'NONE', #48072, #27240, #119535, .T. ) ;
#92555=FACE_BOUND ( 'NONE', #128012, .T. ) ;
#92557=ADVANCED_FACE ( 'NONE', ( #75754 ), #35918, .T. ) ;
#92558=EDGE_CURVE ( 'NONE', #68909, #98740, #25531, .T. ) ;
#92559=CARTESIAN_POINT ( 'NONE',  ( -4.600000000000025402, 2.500000000000000000, 4.430127018922196847 ) ) ;
#92560=CARTESIAN_POINT ( 'NONE',  ( -3.750000000000025757, 12.50000000000000000, 1.472243186433545459 ) ) ;
#92561=CIRCLE ( 'NONE', #52857, 0.06509327318403745899 ) ;
#92562=VERTEX_POINT ( 'NONE', #60019 ) ;
#92563=DIRECTION ( 'NONE',  ( 0.000000000000000000, -0.9999939076577903929, 0.003490651415223739937 ) ) ;
#92564=LINE ( 'NONE', #31718, #78477 ) ;
#92565=CIRCLE ( 'NONE', #103022, 0.1000000000000000056 ) ;
#92566=CIRCLE ( 'NONE', #90501, 0.1000000000000000472 ) ;
#92567=AXIS2_PLACEMENT_3D ( 'NONE', #27544, #39974, #107414 ) ;
#92568=EDGE_CURVE ( 'NONE', #69557, #38337, #38077, .T. ) ;
#92569=LINE ( 'NONE', #44106, #36073 ) ;
#92570=DIRECTION ( 'NONE',  ( 0.000000000000000000, -0.000000000000000000, 1.000000000000000000 ) ) ;
#92571=CARTESIAN_POINT ( 'NONE',  ( 14.19999999999989626, 2.500000000000000000, 0.09999999999999772959 ) ) ;
#92572=EDGE_CURVE ( 'NONE', #59496, #76961, #60653, .T. ) ;
#92573=DIRECTION ( 'NONE',  ( -0.000000000000000000, 1.000000000000000000, -0.000000000000000000 ) ) ;
#92574=AXIS2_PLACEMENT_3D ( 'NONE', #27348, #96737, #56805 ) ;
#92575=PLANE ( 'NONE',  #35779 ) ;
#92577=EDGE_CURVE ( 'NONE', #113875, #16833, #92346, .T. ) ;
#92578=EDGE_LOOP ( 'NONE', ( #34001, #38925, #113662, #15151 ) ) ;
#92579=AXIS2_PLACEMENT_3D ( 'NONE', #1148, #100005, #40455 ) ;
#92580=ORIENTED_EDGE ( 'NONE', *, *, #58801, .T. ) ;
#92581=ORIENTED_EDGE ( 'NONE', *, *, #46156, .T. ) ;
#92582=ORIENTED_EDGE ( 'NONE', *, *, #42961, .F. ) ;
#92583=CARTESIAN_POINT ( 'NONE',  ( 9.149999999999915090, 2.500000000000000000, 6.495190528383297135 ) ) ;
#92585=LINE ( 'NONE', #103037, #40457 ) ;
#92586=ORIENTED_EDGE ( 'NONE', *, *, #56798, .T. ) ;
#92587=FACE_BOUND ( 'NONE', #120703, .T. ) ;
#92588=ADVANCED_FACE ( 'NONE', ( #39089 ), #111210, .T. ) ;
#92589=CARTESIAN_POINT ( 'NONE',  ( -10.85000000000000142, 2.500000000000000000, -2.857883832488649745 ) ) ;
#92590=DIRECTION ( 'NONE',  ( 0.000000000000000000, 0.000000000000000000, 1.000000000000000000 ) ) ;
#92591=CARTESIAN_POINT ( 'NONE',  ( 7.099999999999928590, 2.500000000000000000, 4.230127018922196669 ) ) ;
#92592=DIRECTION ( 'NONE',  ( -0.000000000000000000, -1.000000000000000000, -0.000000000000000000 ) ) ;
#92593=CARTESIAN_POINT ( 'NONE',  ( -6.249999999999981348, 2.500000000000000000, 6.495190528383297135 ) ) ;
#92594=DIRECTION ( 'NONE',  ( -4.274815082592931898E-19, -0.9999939076577903929, -0.003490651415223739937 ) ) ;
#92595=PLANE ( 'NONE',  #116797 ) ;
#92596=CARTESIAN_POINT ( 'NONE',  ( 13.94999999999989271, 2.500000000000000000, -1.818653347947326138 ) ) ;
#92597=AXIS2_PLACEMENT_3D ( 'NONE', #20988, #71363, #19038 ) ;
#92598=DIRECTION ( 'NONE',  ( 0.000000000000000000, -0.000000000000000000, 1.000000000000000000 ) ) ;
#92599=VERTEX_POINT ( 'NONE', #120208 ) ;
#92600=CIRCLE ( 'NONE', #115557, 0.06509327318403745899 ) ;
#92601=VERTEX_POINT ( 'NONE', #99927 ) ;
#92602=EDGE_LOOP ( 'NONE', ( #57043, #2640 ) ) ;
#92603=ORIENTED_EDGE ( 'NONE', *, *, #4896, .T. ) ;
#92604=ORIENTED_EDGE ( 'NONE', *, *, #122178, .F. ) ;
#92605=CIRCLE ( 'NONE', #34117, 0.09999999999999982514 ) ;
#92606=ORIENTED_EDGE ( 'NONE', *, *, #121573, .T. ) ;
#92607=CIRCLE ( 'NONE', #27844, 0.1000000000000002554 ) ;
#92608=FACE_OUTER_BOUND ( 'NONE', #99361, .T. ) ;
#92609=VERTEX_POINT ( 'NONE', #50823 ) ;
#92610=ORIENTED_EDGE ( 'NONE', *, *, #15461, .T. ) ;
#92611=CIRCLE ( 'NONE', #4855, 0.1000000000000002554 ) ;
#92612=CONICAL_SURFACE ( 'NONE', #17366, 0.1000000000000002554, 0.003490658503988666988 ) ;
#92613=CARTESIAN_POINT ( 'NONE',  ( 13.39053294345136003, -2.499999999999999556, 7.037281288959354342 ) ) ;
#92615=DIRECTION ( 'NONE',  ( -0.000000000000000000, 1.000000000000000000, -0.000000000000000000 ) ) ;
#92616=CONICAL_SURFACE ( 'NONE', #109331, 0.09999999999999982514, 0.003490658503988666988 ) ;
#92617=ORIENTED_EDGE ( 'NONE', *, *, #92224, .F. ) ;
#92618=DIRECTION ( 'NONE',  ( 0.000000000000000000, 0.000000000000000000, 1.000000000000000000 ) ) ;
#92619=CIRCLE ( 'NONE', #126055, 0.06509327318403745899 ) ;
#92620=VERTEX_POINT ( 'NONE', #31195 ) ;
#92621=EDGE_CURVE ( 'NONE', #89101, #64737, #8806, .T. ) ;
#92622=VERTEX_POINT ( 'NONE', #89452 ) ;
#92624=EDGE_CURVE ( 'NONE', #20674, #99703, #81984, .T. ) ;
#92626=ORIENTED_EDGE ( 'NONE', *, *, #124594, .T. ) ;
#92627=ORIENTED_EDGE ( 'NONE', *, *, #86531, .F. ) ;
#92628=CONICAL_SURFACE ( 'NONE', #107291, 0.1000000000000002554, 0.003490658503988666988 ) ;
#92629=DIRECTION ( 'NONE',  ( 0.000000000000000000, 1.000000000000000000, 0.000000000000000000 ) ) ;
#92630=CARTESIAN_POINT ( 'NONE',  ( 10.79999999999991012, 12.50000000000000000, 4.395220292106234439 ) ) ;
#92631=DIRECTION ( 'NONE',  ( -0.000000000000000000, 1.000000000000000000, -0.000000000000000000 ) ) ;
#92632=DIRECTION ( 'NONE',  ( 0.000000000000000000, 0.000000000000000000, 1.000000000000000000 ) ) ;
#92633=LINE ( 'NONE', #366, #112970 ) ;
#92634=CONICAL_SURFACE ( 'NONE', #46561, 0.09999999999999999167, 0.003490658503988666988 ) ;
#92635=ORIENTED_EDGE ( 'NONE', *, *, #112791, .T. ) ;
#92636=CARTESIAN_POINT ( 'NONE',  ( 13.54999999999989946, 12.50000000000000000, 2.576566944158910744 ) ) ;
#92637=AXIS2_PLACEMENT_3D ( 'NONE', #122042, #61839, #20617 ) ;
#92638=AXIS2_PLACEMENT_3D ( 'NONE', #41053, #53437, #80959 ) ;
#92639=ORIENTED_EDGE ( 'NONE', *, *, #71291, .T. ) ;
#92640=DIRECTION ( 'NONE',  ( -0.000000000000000000, -1.000000000000000000, -0.000000000000000000 ) ) ;
#92641=ORIENTED_EDGE ( 'NONE', *, *, #22674, .T. ) ;
#92642=DIRECTION ( 'NONE',  ( 0.000000000000000000, 1.000000000000000000, 0.000000000000000000 ) ) ;
#92643=LINE ( 'NONE', #21315, #88662 ) ;
#92644=DIRECTION ( 'NONE',  ( 0.000000000000000000, -0.9999939076577903929, 0.003490651415223739937 ) ) ;
#92646=VECTOR ( 'NONE', #56161, 1000.000000000000000 ) ;
#92647=ORIENTED_EDGE ( 'NONE', *, *, #116288, .F. ) ;
#92648=CONICAL_SURFACE ( 'NONE', #11160, 0.1000000000000002554, 0.003490658503988666988 ) ;
#92649=VECTOR ( 'NONE', #41268, 1000.000000000000000 ) ;
#92650=DIRECTION ( 'NONE',  ( -0.000000000000000000, 1.000000000000000000, -0.000000000000000000 ) ) ;
#92651=AXIS2_PLACEMENT_3D ( 'NONE', #109424, #108129, #119239 ) ;
#92652=DIRECTION ( 'NONE',  ( 0.000000000000000000, 1.000000000000000000, 0.000000000000000000 ) ) ;
#92653=VERTEX_POINT ( 'NONE', #39737 ) ;
#92654=EDGE_LOOP ( 'NONE', ( #21736, #14089, #15209, #15437 ) ) ;
#92655=ORIENTED_EDGE ( 'NONE', *, *, #121688, .T. ) ;
#92656=FACE_OUTER_BOUND ( 'NONE', #117071, .T. ) ;
#92657=DIRECTION ( 'NONE',  ( 0.000000000000000000, 0.000000000000000000, 1.000000000000000000 ) ) ;
#92659=CIRCLE ( 'NONE', #98608, 0.06509327318403741736 ) ;
#92660=CARTESIAN_POINT ( 'NONE',  ( 11.44999999999990692, 2.500000000000000000, 1.718653347947321386 ) ) ;
#92661=CARTESIAN_POINT ( 'NONE',  ( -8.350000000000013856, 2.500000000000000000, -6.395190528383296602 ) ) ;
#92662=ADVANCED_FACE ( 'NONE', ( #111000 ), #96538, .T. ) ;
#92663=DIRECTION ( 'NONE',  ( 0.000000000000000000, 1.000000000000000000, 0.000000000000000000 ) ) ;
#92664=AXIS2_PLACEMENT_3D ( 'NONE', #19274, #100433, #40227 ) ;
#92665=CIRCLE ( 'NONE', #96851, 0.06509327318403745899 ) ;
#92666=AXIS2_PLACEMENT_3D ( 'NONE', #18222, #47708, #88915 ) ;
#92667=CARTESIAN_POINT ( 'NONE',  ( -2.950000000000030376, 2.500000000000000000, 6.595190528383296780 ) ) ;
#92668=CIRCLE ( 'NONE', #126005, 0.1000000000000000056 ) ;
#92669=EDGE_CURVE ( 'NONE', #86369, #125929, #90741, .T. ) ;
#92670=DIRECTION ( 'NONE',  ( 0.000000000000000000, -0.000000000000000000, 1.000000000000000000 ) ) ;
#92671=VERTEX_POINT ( 'NONE', #101212 ) ;
#92672=CARTESIAN_POINT ( 'NONE',  ( -5.800000000000018474, 12.50000000000000000, -2.276824562219559311E-15 ) ) ;
#92673=EDGE_CURVE ( 'NONE', #80874, #13926, #11531, .T. ) ;
#92674=CYLINDRICAL_SURFACE ( 'NONE', #89323, 7.500000000000000000 ) ;
#92675=ADVANCED_FACE ( 'NONE', ( #118910 ), #40139, .T. ) ;
#92676=DIRECTION ( 'NONE',  ( 0.000000000000000000, 0.000000000000000000, -1.000000000000000000 ) ) ;
#92677=DIRECTION ( 'NONE',  ( 0.000000000000000000, 0.000000000000000000, 1.000000000000000000 ) ) ;
#92678=EDGE_LOOP ( 'NONE', ( #119427, #120512 ) ) ;
#92679=DIRECTION ( 'NONE',  ( 0.000000000000000000, 1.000000000000000000, 0.000000000000000000 ) ) ;
#92680=CARTESIAN_POINT ( 'NONE',  ( 1.049999999999954525, 2.500000000000000000, -2.411473670974877859 ) ) ;
#92681=DIRECTION ( 'NONE',  ( -0.000000000000000000, -1.000000000000000000, -0.000000000000000000 ) ) ;
#92682=ORIENTED_EDGE ( 'NONE', *, *, #40588, .F. ) ;
#92683=CONICAL_SURFACE ( 'NONE', #82322, 0.09999999999999982514, 0.003490658503988666988 ) ;
#92684=AXIS2_PLACEMENT_3D ( 'NONE', #39674, #9549, #107079 ) ;
#92685=EDGE_CURVE ( 'NONE', #26619, #8233, #50194, .T. ) ;
#92686=EDGE_LOOP ( 'NONE', ( #122150, #56420, #62738, #38019 ) ) ;
#92688=CIRCLE ( 'NONE', #109414, 0.06509327318403741736 ) ;
#92689=AXIS2_PLACEMENT_3D ( 'NONE', #87487, #127442, #27940 ) ;
#92690=EDGE_LOOP ( 'NONE', ( #118193, #58813 ) ) ;
#92691=AXIS2_PLACEMENT_3D ( 'NONE', #81625, #41733, #39798 ) ;
#92692=EDGE_LOOP ( 'NONE', ( #122269, #52231 ) ) ;
#92693=DIRECTION ( 'NONE',  ( -0.000000000000000000, 1.000000000000000000, -0.000000000000000000 ) ) ;
#92694=AXIS2_PLACEMENT_3D ( 'NONE', #15485, #65231, #55431 ) ;
#92695=AXIS2_PLACEMENT_3D ( 'NONE', #84615, #63693, #15196 ) ;
#92696=PLANE ( 'NONE',  #11234 ) ;
#92697=CARTESIAN_POINT ( 'NONE',  ( 12.49999999999990230, 2.500000000000000000, -0.6928203230275541413 ) ) ;
#92698=CARTESIAN_POINT ( 'NONE',  ( -9.600000000000006750, 2.500000000000000000, 0.6928203230275494784 ) ) ;
#92699=AXIS2_PLACEMENT_3D ( 'NONE', #9134, #127617, #118433 ) ;
#92700=EDGE_LOOP ( 'NONE', ( #66573, #110529, #79760, #25159 ) ) ;
#92701=VECTOR ( 'NONE', #22024, 1000.000000000000000 ) ;
#92702=AXIS2_PLACEMENT_3D ( 'NONE', #93170, #110847, #13288 ) ;
#92703=FACE_OUTER_BOUND ( 'NONE', #83447, .T. ) ;
#92704=DIRECTION ( 'NONE',  ( 0.000000000000000000, 1.000000000000000000, 0.000000000000000000 ) ) ;
#92705=VECTOR ( 'NONE', #85533, 1000.000000000000000 ) ;
#92706=VERTEX_POINT ( 'NONE', #30557 ) ;
#92707=AXIS2_PLACEMENT_3D ( 'NONE', #103604, #15843, #36148 ) ;
#92708=DIRECTION ( 'NONE',  ( 0.000000000000000000, 0.000000000000000000, -1.000000000000000000 ) ) ;
#92709=CARTESIAN_POINT ( 'NONE',  ( 17.45652598566549685, -2.453228361101941424, 4.494719241542497912 ) ) ;
#92710=CIRCLE ( 'NONE', #81942, 0.1000000000000002554 ) ;
#92711=ORIENTED_EDGE ( 'NONE', *, *, #50638, .T. ) ;
#92712=ADVANCED_FACE ( 'NONE', ( #29260 ), #69361, .T. ) ;
#92713=ORIENTED_EDGE ( 'NONE', *, *, #79725, .T. ) ;
#92714=EDGE_LOOP ( 'NONE', ( #57158, #46248 ) ) ;
#92715=ORIENTED_EDGE ( 'NONE', *, *, #97151, .T. ) ;
#92716=CARTESIAN_POINT ( 'NONE',  ( 12.04999999999990479, 12.50000000000000000, -6.495190528383302464 ) ) ;
#92717=CARTESIAN_POINT ( 'NONE',  ( 15.50668943717079351, 1.500000000000191847, 6.997696160023704870 ) ) ;
#92718=DIRECTION ( 'NONE',  ( 0.000000000000000000, -0.9999939076577903929, 0.003490651415223739937 ) ) ;
#92719=ADVANCED_FACE ( 'NONE', ( #111678 ), #79010, .T. ) ;
#92720=FACE_BOUND ( 'NONE', #33935, .T. ) ;
#92721=EDGE_LOOP ( 'NONE', ( #18398, #35557, #35794, #102212 ) ) ;
#92723=EDGE_CURVE ( 'NONE', #104908, #63527, #109055, .T. ) ;
#92724=DIRECTION ( 'NONE',  ( 0.000000000000000000, 0.000000000000000000, -1.000000000000000000 ) ) ;
#92725=DIRECTION ( 'NONE',  ( -0.000000000000000000, 1.000000000000000000, -0.000000000000000000 ) ) ;
#92726=AXIS2_PLACEMENT_3D ( 'NONE', #94972, #115211, #106074 ) ;
#92727=ADVANCED_FACE ( 'NONE', ( #9602 ), #49545, .T. ) ;
#92729=EDGE_CURVE ( 'NONE', #63286, #89688, #53403, .T. ) ;
#92730=CARTESIAN_POINT ( 'NONE',  ( -8.150000000000012790, 2.500000000000000000, 2.611473670974873151 ) ) ;
#92731=ADVANCED_FACE ( 'NONE', ( #23944 ), #4267, .T. ) ;
#92732=CARTESIAN_POINT ( 'NONE',  ( 1.899999999999951283, 2.500000000000000000, 0.2464101615137736789 ) ) ;
#92733=CIRCLE ( 'NONE', #78055, 0.09999999999999982514 ) ;
#92734=AXIS2_PLACEMENT_3D ( 'NONE', #64870, #33510, #23673 ) ;
#92735=VECTOR ( 'NONE', #2059, 1000.000000000000000 ) ;
#92736=DIRECTION ( 'NONE',  ( -0.000000000000000000, -1.000000000000000000, -0.000000000000000000 ) ) ;
#92737=ADVANCED_FACE ( 'NONE', ( #13459 ), #88212, .T. ) ;
#92738=ORIENTED_EDGE ( 'NONE', *, *, #85283, .T. ) ;
#92739=VERTEX_POINT ( 'NONE', #74325 ) ;
#92740=VERTEX_POINT ( 'NONE', #84785 ) ;
#92741=ORIENTED_EDGE ( 'NONE', *, *, #64943, .F. ) ;
#92742=ORIENTED_EDGE ( 'NONE', *, *, #1864, .T. ) ;
#92743=CARTESIAN_POINT ( 'NONE',  ( 6.049999999999932321, 12.50000000000000000, 1.818653347947321475 ) ) ;
#92744=LINE ( 'NONE', #24000, #107236 ) ;
#92746=FACE_BOUND ( 'NONE', #21470, .T. ) ;
#92747=AXIS2_PLACEMENT_3D ( 'NONE', #18821, #49598, #118959 ) ;
#92748=CIRCLE ( 'NONE', #50785, 0.06509327318403745899 ) ;
#92749=EDGE_CURVE ( 'NONE', #98360, #127025, #123729, .T. ) ;
#92750=DIRECTION ( 'NONE',  ( 0.000000000000000000, -0.000000000000000000, 1.000000000000000000 ) ) ;
#92751=VECTOR ( 'NONE', #91634, 1000.000000000000000 ) ;
#92752=VECTOR ( 'NONE', #26200, 1000.000000000000000 ) ;
#92753=EDGE_LOOP ( 'NONE', ( #15444, #56401, #76565, #67248 ) ) ;
#92754=DIRECTION ( 'NONE',  ( 0.000000000000000000, 0.000000000000000000, -1.000000000000000000 ) ) ;
#92755=PLANE ( 'NONE',  #5159 ) ;
#92757=CONICAL_SURFACE ( 'NONE', #46792, 0.1000000000000000472, 0.003490658503988666988 ) ;
#92758=ORIENTED_EDGE ( 'NONE', *, *, #64843, .F. ) ;
#92759=DIRECTION ( 'NONE',  ( -0.000000000000000000, -1.000000000000000000, -0.000000000000000000 ) ) ;
#92760=EDGE_LOOP ( 'NONE', ( #79564, #47263 ) ) ;
#92761=CIRCLE ( 'NONE', #36346, 0.06509327318403745899 ) ;
#92762=AXIS2_PLACEMENT_3D ( 'NONE', #101445, #51704, #72634 ) ;
#92763=AXIS2_PLACEMENT_3D ( 'NONE', #93423, #44313, #84230 ) ;
#92764=EDGE_LOOP ( 'NONE', ( #95332, #56465, #117401, #45563 ) ) ;
#92766=DIRECTION ( 'NONE',  ( 0.000000000000000000, -0.000000000000000000, 1.000000000000000000 ) ) ;
#92767=PLANE ( 'NONE',  #108261 ) ;
#92768=CARTESIAN_POINT ( 'NONE',  ( -12.04999999999999538, 12.50000000000000000, 2.165063509461097713 ) ) ;
#92769=VECTOR ( 'NONE', #53316, 1000.000000000000000 ) ;
#92770=ORIENTED_EDGE ( 'NONE', *, *, #71849, .T. ) ;
#92771=CARTESIAN_POINT ( 'NONE',  ( 6.899999999999928413, 2.500000000000000000, -3.983716857408426293 ) ) ;
#92772=AXIS2_PLACEMENT_3D ( 'NONE', #119281, #28989, #68247 ) ;
#92773=DIRECTION ( 'NONE',  ( 0.000000000000000000, -0.9999939076577903929, 0.003490651415223739937 ) ) ;
#92774=DIRECTION ( 'NONE',  ( 0.000000000000000000, 0.000000000000000000, -1.000000000000000000 ) ) ;
#92776=VERTEX_POINT ( 'NONE', #44880 ) ;
#92777=CARTESIAN_POINT ( 'NONE',  ( 3.099999999999945466, 12.50000000000000000, 0.3464101615137735735 ) ) ;
#92778=ORIENTED_EDGE ( 'NONE', *, *, #67229, .F. ) ;
#92779=PLANE ( 'NONE',  #86789 ) ;
#92780=ORIENTED_EDGE ( 'NONE', *, *, #116340, .T. ) ;
#92782=ORIENTED_EDGE ( 'NONE', *, *, #64792, .F. ) ;
#92784=CARTESIAN_POINT ( 'NONE',  ( 2.899999999999945732, 2.500000000000000000, -4.330127018922201643 ) ) ;
#92785=VECTOR ( 'NONE', #21481, 1000.000000000000000 ) ;
#92786=CARTESIAN_POINT ( 'NONE',  ( 8.949999999999919353, 2.500000000000000000, -6.248780366869526759 ) ) ;
#92787=CIRCLE ( 'NONE', #32160, 0.06509327318403745899 ) ;
#92788=CARTESIAN_POINT ( 'NONE',  ( 14.34999999999989662, 12.50000000000000000, 2.511473670974873507 ) ) ;
#92789=DIRECTION ( 'NONE',  ( -4.274815082592931898E-19, -0.9999939076577903929, -0.003490651415223739937 ) ) ;
#92790=ORIENTED_EDGE ( 'NONE', *, *, #77364, .T. ) ;
#92791=EDGE_LOOP ( 'NONE', ( #19720, #30704, #18487, #111026 ) ) ;
#92792=EDGE_CURVE ( 'NONE', #15955, #28223, #12914, .T. ) ;
#92794=AXIS2_PLACEMENT_3D ( 'NONE', #90597, #112828, #23149 ) ;
#92795=AXIS2_PLACEMENT_3D ( 'NONE', #110366, #61278, #101200 ) ;
#92796=CIRCLE ( 'NONE', #23836, 0.06509327318403741736 ) ;
#92797=LINE ( 'NONE', #113057, #24347 ) ;
#92798=AXIS2_PLACEMENT_3D ( 'NONE', #83465, #65071, #18412 ) ;
#92799=AXIS2_PLACEMENT_3D ( 'NONE', #14566, #105548, #34245 ) ;
#92800=DIRECTION ( 'NONE',  ( 0.000000000000000000, 0.000000000000000000, -1.000000000000000000 ) ) ;
#92801=VERTEX_POINT ( 'NONE', #42291 ) ;
#92802=EDGE_LOOP ( 'NONE', ( #48398, #114639 ) ) ;
#92803=FACE_OUTER_BOUND ( 'NONE', #87366, .T. ) ;
#92804=EDGE_LOOP ( 'NONE', ( #85361, #63958 ) ) ;
#92805=CARTESIAN_POINT ( 'NONE',  ( 0.3999999999999563904, 2.500000000000000000, 5.022947341949748790 ) ) ;
#92806=CARTESIAN_POINT ( 'NONE',  ( -6.450000000000016165, 2.500000000000000000, 2.511473670974873507 ) ) ;
#92807=CIRCLE ( 'NONE', #21800, 0.1000000000000002554 ) ;
#92808=AXIS2_PLACEMENT_3D ( 'NONE', #54459, #45306, #85209 ) ;
#92809=AXIS2_PLACEMENT_3D ( 'NONE', #9984, #99008, #68897 ) ;
#92810=DIRECTION ( 'NONE',  ( 0.000000000000000000, -0.9999939076577903929, 0.003490651415223739937 ) ) ;
#92811=EDGE_LOOP ( 'NONE', ( #17236, #67457 ) ) ;
#92812=CARTESIAN_POINT ( 'NONE',  ( -9.800000000000007816, 2.500000000000000000, -3.983716857408421852 ) ) ;
#92813=CARTESIAN_POINT ( 'NONE',  ( -5.650000000000019895, 2.500000000000000000, 6.841600689897072485 ) ) ;
#92814=DIRECTION ( 'NONE',  ( 0.000000000000000000, 1.000000000000000000, 0.000000000000000000 ) ) ;
#92815=LINE ( 'NONE', #73165, #42625 ) ;
#92816=AXIS2_PLACEMENT_3D ( 'NONE', #33425, #24877, #43889 ) ;
#92817=CARTESIAN_POINT ( 'NONE',  ( -11.64999999999999680, 2.500000000000000000, -7.188010851410850499 ) ) ;
#92818=VERTEX_POINT ( 'NONE', #124063 ) ;
#92819=CARTESIAN_POINT ( 'NONE',  ( 6.649999999999928413, 12.50000000000000000, 2.922977105672686982 ) ) ;
#92820=DIRECTION ( 'NONE',  ( 0.000000000000000000, 0.000000000000000000, 1.000000000000000000 ) ) ;
#92822=VERTEX_POINT ( 'NONE', #103785 ) ;
#92824=DIRECTION ( 'NONE',  ( -4.274815082592931898E-19, -0.9999939076577903929, -0.003490651415223739937 ) ) ;
#92825=CARTESIAN_POINT ( 'NONE',  ( 13.34999999999989662, 2.500000000000000000, -2.165063509461101710 ) ) ;
#92826=CONICAL_SURFACE ( 'NONE', #36396, 0.1000000000000002554, 0.003490658503988666988 ) ;
#92827=CARTESIAN_POINT ( 'NONE',  ( -5.650000000000019895, 2.500000000000000000, 6.841600689897072485 ) ) ;
#92828=DIRECTION ( 'NONE',  ( 0.000000000000000000, 1.000000000000000000, 0.000000000000000000 ) ) ;
#92829=EDGE_CURVE ( 'NONE', #9926, #110798, #56821, .T. ) ;
#92830=DIRECTION ( 'NONE',  ( 0.000000000000000000, 0.000000000000000000, 1.000000000000000000 ) ) ;
#92831=DIRECTION ( 'NONE',  ( 0.000000000000000000, 0.000000000000000000, 1.000000000000000000 ) ) ;
#92833=DIRECTION ( 'NONE',  ( 0.000000000000000000, 0.000000000000000000, 1.000000000000000000 ) ) ;
#92834=CARTESIAN_POINT ( 'NONE',  ( 12.49999999999990052, 2.500000000000000000, 0.6928203230275494784 ) ) ;
#92835=EDGE_CURVE ( 'NONE', #15358, #56070, #124712, .T. ) ;
#92836=EDGE_LOOP ( 'NONE', ( #88384, #35759, #23630, #62519 ) ) ;
#92837=CIRCLE ( 'NONE', #38462, 0.06509327318403745899 ) ;
#92838=EDGE_LOOP ( 'NONE', ( #103405, #102519, #28812, #4007 ) ) ;
#92839=EDGE_LOOP ( 'NONE', ( #71536, #34853 ) ) ;
#92840=EDGE_CURVE ( 'NONE', #56576, #51026, #19178, .T. ) ;
#92841=ORIENTED_EDGE ( 'NONE', *, *, #29625, .T. ) ;
#92842=AXIS2_PLACEMENT_3D ( 'NONE', #73713, #11580, #10908 ) ;
#92843=ADVANCED_FACE ( 'NONE', ( #33752 ), #35062, .T. ) ;
#92844=DIRECTION ( 'NONE',  ( 0.000000000000000000, -0.000000000000000000, 1.000000000000000000 ) ) ;
#92846=CIRCLE ( 'NONE', #36417, 0.09999999999999982514 ) ;
#92847=VERTEX_POINT ( 'NONE', #32494 ) ;
#92848=CARTESIAN_POINT ( 'NONE',  ( -5.600000000000023626, 2.500000000000000000, -4.676537180435977881 ) ) ;
#92850=DIRECTION ( 'NONE',  ( 0.000000000000000000, 0.000000000000000000, 1.000000000000000000 ) ) ;
#92852=ORIENTED_EDGE ( 'NONE', *, *, #44811, .T. ) ;
#92853=EDGE_CURVE ( 'NONE', #114323, #103313, #46371, .T. ) ;
#92854=CARTESIAN_POINT ( 'NONE',  ( 5.849999999999933920, 12.50000000000000000, -2.792790559304616504 ) ) ;
#92855=PLANE ( 'NONE',  #79307 ) ;
#92856=VERTEX_POINT ( 'NONE', #114245 ) ;
#92857=AXIS2_PLACEMENT_3D ( 'NONE', #9966, #93045, #112037 ) ;
#92858=AXIS2_PLACEMENT_3D ( 'NONE', #42543, #121080, #71319 ) ;
#92859=CONICAL_SURFACE ( 'NONE', #122103, 0.09999999999999982514, 0.003490658503988666988 ) ;
#92860=ORIENTED_EDGE ( 'NONE', *, *, #97344, .T. ) ;
#92861=ORIENTED_EDGE ( 'NONE', *, *, #105700, .T. ) ;
#92862=VERTEX_POINT ( 'NONE', #114879 ) ;
#92863=DIRECTION ( 'NONE',  ( -0.000000000000000000, -1.000000000000000000, -0.000000000000000000 ) ) ;
#92864=VECTOR ( 'NONE', #106899, 1000.000000000000000 ) ;
#92865=CARTESIAN_POINT ( 'NONE',  ( 8.299999999999922551, 2.500000000000000000, -4.430127018922202176 ) ) ;
#92866=DIRECTION ( 'NONE',  ( 0.000000000000000000, 1.000000000000000000, 0.000000000000000000 ) ) ;
#92867=CIRCLE ( 'NONE', #36441, 0.09999999999999999167 ) ;
#92868=DIRECTION ( 'NONE',  ( 0.000000000000000000, 1.000000000000000000, 0.000000000000000000 ) ) ;
#92869=VERTEX_POINT ( 'NONE', #65126 ) ;
#92870=PLANE ( 'NONE',  #58569 ) ;
#92871=EDGE_LOOP ( 'NONE', ( #111214, #23951, #101091, #49701 ) ) ;
#92873=DIRECTION ( 'NONE',  ( -0.000000000000000000, -1.000000000000000000, -0.000000000000000000 ) ) ;
#92874=CARTESIAN_POINT ( 'NONE',  ( -9.800000000000004263, 12.50000000000000000, 3.983716857408420076 ) ) ;
#92875=CARTESIAN_POINT ( 'NONE',  ( -2.100000000000033396, 12.50000000000000000, -0.6928203230275542523 ) ) ;
#92876=ORIENTED_EDGE ( 'NONE', *, *, #119772, .T. ) ;
#92878=ORIENTED_EDGE ( 'NONE', *, *, #23124, .F. ) ;
#92879=CONICAL_SURFACE ( 'NONE', #30191, 0.09999999999999982514, 0.003490658503988666988 ) ;
#92880=ORIENTED_EDGE ( 'NONE', *, *, #94273, .F. ) ;
#92881=CARTESIAN_POINT ( 'NONE',  ( -0.8500000000000386136, 2.500000000000000000, 5.802370205355744659 ) ) ;
#92882=CARTESIAN_POINT ( 'NONE',  ( -11.05000000000000071, 2.500000000000000000, 2.611473670974873151 ) ) ;
#92883=CONICAL_SURFACE ( 'NONE', #86593, 0.09999999999999982514, 0.003490658503988666988 ) ;
#92885=CARTESIAN_POINT ( 'NONE',  ( -11.24999999999996270, 2.500000000000000000, 6.495190528383297135 ) ) ;
#92886=FACE_BOUND ( 'NONE', #26680, .T. ) ;
#92887=DIRECTION ( 'NONE',  ( -0.000000000000000000, 1.000000000000000000, -0.000000000000000000 ) ) ;
#92888=DIRECTION ( 'NONE',  ( 0.000000000000000000, -0.9999939076577903929, 0.003490651415223739937 ) ) ;
#92889=EDGE_CURVE ( 'NONE', #129244, #60586, #84027, .T. ) ;
#92890=DIRECTION ( 'NONE',  ( 0.000000000000000000, 0.000000000000000000, -1.000000000000000000 ) ) ;
#92891=AXIS2_PLACEMENT_3D ( 'NONE', #99632, #62132, #79979 ) ;
#92892=AXIS2_PLACEMENT_3D ( 'NONE', #46010, #124568, #115352 ) ;
#92893=ADVANCED_FACE ( 'NONE', ( #12162 ), #42965, .T. ) ;
#92894=EDGE_CURVE ( 'NONE', #115059, #85204, #82867, .T. ) ;
#92897=EDGE_CURVE ( 'NONE', #71057, #102543, #5562, .T. ) ;
#92898=CARTESIAN_POINT ( 'NONE',  ( 14.99999999999992895, 2.500000000000000000, -2.276824562219559311E-15 ) ) ;
#92899=ORIENTED_EDGE ( 'NONE', *, *, #119486, .T. ) ;
#92900=ADVANCED_FACE ( 'NONE', ( #17301 ), #31912, .T. ) ;
#92901=VECTOR ( 'NONE', #127464, 1000.000000000000000 ) ;
#92902=AXIS2_PLACEMENT_3D ( 'NONE', #37906, #19559, #59517 ) ;
#92903=AXIS2_PLACEMENT_3D ( 'NONE', #39325, #118484, #28839 ) ;
#92904=DIRECTION ( 'NONE',  ( 0.000000000000000000, -0.000000000000000000, 1.000000000000000000 ) ) ;
#92905=EDGE_CURVE ( 'NONE', #123229, #126098, #29755, .T. ) ;
#92906=ORIENTED_EDGE ( 'NONE', *, *, #101700, .F. ) ;
#92907=VERTEX_POINT ( 'NONE', #56595 ) ;
#92908=AXIS2_PLACEMENT_3D ( 'NONE', #70602, #81074, #20856 ) ;
#92909=CARTESIAN_POINT ( 'NONE',  ( -3.750000000000029310, 2.500000000000000000, -7.188010851410854052 ) ) ;
#92910=FACE_OUTER_BOUND ( 'NONE', #69823, .T. ) ;
#92911=FACE_BOUND ( 'NONE', #10730, .T. ) ;
#92912=CARTESIAN_POINT ( 'NONE',  ( -5.800000000000018474, 2.500000000000000000, -2.276824562219559311E-15 ) ) ;
#92913=ADVANCED_FACE ( 'NONE', ( #57266 ), #59100, .T. ) ;
#92914=EDGE_CURVE ( 'NONE', #79722, #65565, #77860, .T. ) ;
#92915=VERTEX_POINT ( 'NONE', #97186 ) ;
#92916=CARTESIAN_POINT ( 'NONE',  ( 81.97620568553573150, 3.937821662797851729, 6.124242991678374715 ) ) ;
#92917=DIRECTION ( 'NONE',  ( 0.000000000000000000, 0.000000000000000000, 1.000000000000000000 ) ) ;
#92918=AXIS2_PLACEMENT_3D ( 'NONE', #53864, #13920, #55793 ) ;
#92919=VERTEX_POINT ( 'NONE', #67713 ) ;
#92920=DIRECTION ( 'NONE',  ( 0.000000000000000000, -0.9999939076577903929, 0.003490651415223739937 ) ) ;
#92921=CARTESIAN_POINT ( 'NONE',  ( -7.900000000000014566, 12.50000000000000000, -4.330127018922201643 ) ) ;
#92922=ORIENTED_EDGE ( 'NONE', *, *, #42957, .T. ) ;
#92923=CARTESIAN_POINT ( 'NONE',  ( -8.749999999999976907, 12.50000000000000000, -6.430097255199259010 ) ) ;
#92924=DIRECTION ( 'NONE',  ( -0.000000000000000000, -1.000000000000000000, -0.000000000000000000 ) ) ;
#92925=CIRCLE ( 'NONE', #84602, 0.06509327318403745899 ) ;
#92926=CIRCLE ( 'NONE', #40711, 0.09999999999999982514 ) ;
#92927=ORIENTED_EDGE ( 'NONE', *, *, #127694, .T. ) ;
#92928=DIRECTION ( 'NONE',  ( 0.000000000000000000, 0.000000000000000000, 1.000000000000000000 ) ) ;
#92929=CARTESIAN_POINT ( 'NONE',  ( 1.699999999999951994, 2.500000000000000000, -2.276824562219559311E-15 ) ) ;
#92930=DIRECTION ( 'NONE',  ( 0.000000000000000000, 0.000000000000000000, 1.000000000000000000 ) ) ;
#92931=ORIENTED_EDGE ( 'NONE', *, *, #120436, .T. ) ;
#92932=EDGE_LOOP ( 'NONE', ( #97419, #25790 ) ) ;
#92933=CARTESIAN_POINT ( 'NONE',  ( 9.799999999999917222, 12.50000000000000000, 0.2813168883297361700 ) ) ;
#92934=VERTEX_POINT ( 'NONE', #16663 ) ;
#92935=CARTESIAN_POINT ( 'NONE',  ( 4.599999999999938360, 12.50000000000000000, -0.6928203230275541413 ) ) ;
#92936=DIRECTION ( 'NONE',  ( -0.000000000000000000, 1.000000000000000000, -0.000000000000000000 ) ) ;
#92937=CIRCLE ( 'NONE', #69947, 0.1000000000000002554 ) ;
#92939=AXIS2_PLACEMENT_3D ( 'NONE', #55701, #54411, #85801 ) ;
#92940=DIRECTION ( 'NONE',  ( 0.000000000000000000, -0.000000000000000000, 1.000000000000000000 ) ) ;
#92941=DIRECTION ( 'NONE',  ( 0.000000000000000000, -0.000000000000000000, 1.000000000000000000 ) ) ;
#92942=DIRECTION ( 'NONE',  ( -0.000000000000000000, -1.000000000000000000, -0.000000000000000000 ) ) ;
#92943=FACE_OUTER_BOUND ( 'NONE', #72219, .T. ) ;
#92944=CARTESIAN_POINT ( 'NONE',  ( 6.699999999999930012, 12.50000000000000000, -4.395220292106239768 ) ) ;
#92945=ORIENTED_EDGE ( 'NONE', *, *, #34924, .F. ) ;
#92946=ADVANCED_FACE ( 'NONE', ( #45522 ), #88315, .T. ) ;
#92947=ORIENTED_EDGE ( 'NONE', *, *, #862, .F. ) ;
#92948=DIRECTION ( 'NONE',  ( -0.000000000000000000, -1.000000000000000000, -0.000000000000000000 ) ) ;
#92949=CONICAL_SURFACE ( 'NONE', #36518, 0.1000000000000000472, 0.003490658503988666988 ) ;
#92950=VERTEX_POINT ( 'NONE', #87347 ) ;
#92951=AXIS2_PLACEMENT_3D ( 'NONE', #46875, #125425, #35758 ) ;
#92952=CARTESIAN_POINT ( 'NONE',  ( -8.550000000000013145, 12.50000000000000000, 2.511473670974873507 ) ) ;
#92953=EDGE_LOOP ( 'NONE', ( #21319, #128799 ) ) ;
#92954=EDGE_LOOP ( 'NONE', ( #68826, #113588 ) ) ;
#92955=VERTEX_POINT ( 'NONE', #47447 ) ;
#92956=CIRCLE ( 'NONE', #67803, 0.06509327318403741736 ) ;
#92957=PLANE ( 'NONE',  #114796 ) ;
#92958=CIRCLE ( 'NONE', #65744, 0.06509327318403745899 ) ;
#92959=FACE_OUTER_BOUND ( 'NONE', #108557, .T. ) ;
#92960=FACE_OUTER_BOUND ( 'NONE', #76589, .T. ) ;
#92962=DIRECTION ( 'NONE',  ( 0.000000000000000000, 0.000000000000000000, 1.000000000000000000 ) ) ;
#92963=DIRECTION ( 'NONE',  ( -0.000000000000000000, 1.000000000000000000, -0.000000000000000000 ) ) ;
#92964=CARTESIAN_POINT ( 'NONE',  ( -4.550000000000022915, 2.500000000000000000, 2.165063509461097713 ) ) ;
#92965=CARTESIAN_POINT ( 'NONE',  ( 4.399999999999937295, 12.50000000000000000, 3.983716857408420964 ) ) ;
#92966=DIRECTION ( 'NONE',  ( 0.000000000000000000, 0.000000000000000000, 1.000000000000000000 ) ) ;
#92967=DIRECTION ( 'NONE',  ( 0.000000000000000000, -0.000000000000000000, 1.000000000000000000 ) ) ;
#92968=ORIENTED_EDGE ( 'NONE', *, *, #95830, .F. ) ;
#92969=AXIS2_PLACEMENT_3D ( 'NONE', #120196, #99272, #60641 ) ;
#92970=DIRECTION ( 'NONE',  ( 0.000000000000000000, 1.000000000000000000, 0.000000000000000000 ) ) ;
#92971=CIRCLE ( 'NONE', #3083, 0.06509327318403745899 ) ;
#92972=CIRCLE ( 'NONE', #61671, 0.06509327318403745899 ) ;
#92973=ORIENTED_EDGE ( 'NONE', *, *, #4742, .T. ) ;
#92975=CARTESIAN_POINT ( 'NONE',  ( 5.849999999999931255, 12.50000000000000000, 2.792790559304612064 ) ) ;
#92976=CARTESIAN_POINT ( 'NONE',  ( 0.5999999999999612310, 2.500000000000000000, -0.3464101615137760715 ) ) ;
#92977=LINE ( 'NONE', #100832, #79988 ) ;
#92978=AXIS2_PLACEMENT_3D ( 'NONE', #34543, #53524, #33866 ) ;
#92979=DIRECTION ( 'NONE',  ( 0.000000000000000000, 1.000000000000000000, 0.000000000000000000 ) ) ;
#92980=AXIS2_PLACEMENT_3D ( 'NONE', #129218, #37597, #59836 ) ;
#92981=CARTESIAN_POINT ( 'NONE',  ( 5.649999999999934630, 12.50000000000000000, -2.511473670974877948 ) ) ;
#92982=FACE_OUTER_BOUND ( 'NONE', #74969, .T. ) ;
#92983=PLANE ( 'NONE',  #122053 ) ;
#92984=EDGE_LOOP ( 'NONE', ( #65519, #75468, #85548, #97303 ) ) ;
#92985=VECTOR ( 'NONE', #10234, 1000.000000000000000 ) ;
#92986=ORIENTED_EDGE ( 'NONE', *, *, #91656, .F. ) ;
#92987=CIRCLE ( 'NONE', #126439, 0.06509327318403745899 ) ;
#92988=EDGE_CURVE ( 'NONE', #98668, #125752, #106987, .T. ) ;
#92989=ORIENTED_EDGE ( 'NONE', *, *, #121633, .F. ) ;
#92990=VERTEX_POINT ( 'NONE', #127302 ) ;
#92991=VECTOR ( 'NONE', #94742, 1000.000000000000000 ) ;
#92992=EDGE_CURVE ( 'NONE', #66128, #16718, #96516, .T. ) ;
#92993=ORIENTED_EDGE ( 'NONE', *, *, #38153, .F. ) ;
#92994=EDGE_CURVE ( 'NONE', #67445, #3107, #8902, .T. ) ;
#92995=FACE_OUTER_BOUND ( 'NONE', #23126, .T. ) ;
#92996=CARTESIAN_POINT ( 'NONE',  ( -1.700000000000034817, 2.500000000000000000, -4.330127018922201643 ) ) ;
#92997=LINE ( 'NONE', #73333, #79903 ) ;
#92998=PLANE ( 'NONE',  #123881 ) ;
#92999=EDGE_CURVE ( 'NONE', #62494, #10784, #27681, .T. ) ;
#93000=DIRECTION ( 'NONE',  ( 0.000000000000000000, 0.000000000000000000, 1.000000000000000000 ) ) ;
#93001=ADVANCED_FACE ( 'NONE', ( #35696 ), #21434, .T. ) ;
#93002=VERTEX_POINT ( 'NONE', #57919 ) ;
#93003=CARTESIAN_POINT ( 'NONE',  ( 65.39894239681107990, -3.129862336044758386, 5.811320851586441627 ) ) ;
#93004=EDGE_CURVE ( 'NONE', #23771, #17021, #19364, .T. ) ;
#93005=CARTESIAN_POINT ( 'NONE',  ( 11.64999999999990443, 12.50000000000000000, -7.188010851410854052 ) ) ;
#93006=EDGE_CURVE ( 'NONE', #844, #101014, #61152, .T. ) ;
#93007=CARTESIAN_POINT ( 'NONE',  ( 7.949999999999922018, 12.50000000000000000, -2.165063509461101710 ) ) ;
#93008=AXIS2_PLACEMENT_3D ( 'NONE', #97091, #105630, #56513 ) ;
#93009=DIRECTION ( 'NONE',  ( 0.000000000000000000, 0.000000000000000000, 1.000000000000000000 ) ) ;
#93011=ORIENTED_EDGE ( 'NONE', *, *, #52512, .F. ) ;
#93012=VERTEX_POINT ( 'NONE', #105053 ) ;
#93013=CARTESIAN_POINT ( 'NONE',  ( 5.399999999999933742, 12.50000000000000000, -0.06509327318403980434 ) ) ;
#93015=AXIS2_PLACEMENT_3D ( 'NONE', #3567, #81491, #83432 ) ;
#93016=DIRECTION ( 'NONE',  ( 0.000000000000000000, 0.000000000000000000, -1.000000000000000000 ) ) ;
#93017=DIRECTION ( 'NONE',  ( 0.000000000000000000, -0.9999939076577903929, 0.003490651415223739937 ) ) ;
#93018=VERTEX_POINT ( 'NONE', #55960 ) ;
#93019=CARTESIAN_POINT ( 'NONE',  ( -7.700000000000010836, 2.500000000000000000, 3.983716857408420964 ) ) ;
#93020=DIRECTION ( 'NONE',  ( -0.000000000000000000, 1.000000000000000000, -0.000000000000000000 ) ) ;
#93021=DIRECTION ( 'NONE',  ( 0.000000000000000000, 1.000000000000000000, 0.000000000000000000 ) ) ;
#93022=LINE ( 'NONE', #60969, #70616 ) ;
#93023=AXIS2_PLACEMENT_3D ( 'NONE', #55830, #17831, #78047 ) ;
#93024=CARTESIAN_POINT ( 'NONE',  ( 4.149999999999941735, 2.500000000000000000, -7.288010851410854585 ) ) ;
#93025=VERTEX_POINT ( 'NONE', #95898 ) ;
#93026=ORIENTED_EDGE ( 'NONE', *, *, #10659, .T. ) ;
#93027=ADVANCED_FACE ( 'NONE', ( #6204 ), #36356, .T. ) ;
#93029=CARTESIAN_POINT ( 'NONE',  ( -9.150000000000005684, 12.50000000000000000, 5.867463478539781896 ) ) ;
#93030=DIRECTION ( 'NONE',  ( -0.000000000000000000, 1.000000000000000000, -0.000000000000000000 ) ) ;
#93031=DIRECTION ( 'NONE',  ( 0.000000000000000000, 0.000000000000000000, -1.000000000000000000 ) ) ;
#93032=DIRECTION ( 'NONE',  ( -0.000000000000000000, 1.000000000000000000, -0.000000000000000000 ) ) ;
#93033=ORIENTED_EDGE ( 'NONE', *, *, #30997, .T. ) ;
#93034=VECTOR ( 'NONE', #986, 1000.000000000000000 ) ;
#93035=EDGE_CURVE ( 'NONE', #49015, #70759, #102910, .T. ) ;
#93036=ORIENTED_EDGE ( 'NONE', *, *, #124805, .F. ) ;
#93037=EDGE_CURVE ( 'NONE', #120364, #18875, #92535, .T. ) ;
#93038=LINE ( 'NONE', #64847, #83620 ) ;
#93039=DIRECTION ( 'NONE',  ( 0.000000000000000000, 1.000000000000000000, 0.000000000000000000 ) ) ;
#93040=CARTESIAN_POINT ( 'NONE',  ( -1.450000000000035483, 12.50000000000000000, 6.148780366869520897 ) ) ;
#93041=DIRECTION ( 'NONE',  ( 0.000000000000000000, 0.000000000000000000, 1.000000000000000000 ) ) ;
#93042=ADVANCED_FACE ( 'NONE', ( #81425 ), #111298, .T. ) ;
#93043=CARTESIAN_POINT ( 'NONE',  ( -6.450000000000019718, 2.500000000000000000, -6.148780366869526226 ) ) ;
#93044=ORIENTED_EDGE ( 'NONE', *, *, #95095, .F. ) ;
#93045=DIRECTION ( 'NONE',  ( -0.000000000000000000, 1.000000000000000000, -0.000000000000000000 ) ) ;
#93046=EDGE_CURVE ( 'NONE', #16038, #102251, #40208, .T. ) ;
#93047=DIRECTION ( 'NONE',  ( 0.000000000000000000, 0.000000000000000000, -1.000000000000000000 ) ) ;
#93048=ORIENTED_EDGE ( 'NONE', *, *, #115979, .F. ) ;
#93049=DIRECTION ( 'NONE',  ( -4.274815082592931898E-19, -0.9999939076577903929, -0.003490651415223739937 ) ) ;
#93050=EDGE_CURVE ( 'NONE', #17558, #95927, #60505, .T. ) ;
#93051=AXIS2_PLACEMENT_3D ( 'NONE', #35968, #24218, #105352 ) ;
#93052=EDGE_LOOP ( 'NONE', ( #68478, #114986, #129269, #81704 ) ) ;
#93053=CARTESIAN_POINT ( 'NONE',  ( -3.469446951953614189E-14, 2.500000000000000000, -0.5928203230275518321 ) ) ;
#93054=ADVANCED_FACE ( 'NONE', ( #59871 ), #38165, .T. ) ;
#93055=EDGE_CURVE ( 'NONE', #117313, #46303, #52736, .T. ) ;
#93056=ADVANCED_FACE ( 'NONE', ( #50664 ), #88654, .T. ) ;
#93057=AXIS2_PLACEMENT_3D ( 'NONE', #31115, #61856, #52034 ) ;
#93058=EDGE_LOOP ( 'NONE', ( #82853, #15741, #47337, #9287 ) ) ;
#93059=DIRECTION ( 'NONE',  ( 0.000000000000000000, 1.000000000000000000, 0.000000000000000000 ) ) ;
#93060=DIRECTION ( 'NONE',  ( -0.000000000000000000, -1.000000000000000000, -0.000000000000000000 ) ) ;
#93061=AXIS2_PLACEMENT_3D ( 'NONE', #8766, #20550, #244 ) ;
#93062=CONICAL_SURFACE ( 'NONE', #61770, 0.09999999999999982514, 0.003490658503988666988 ) ;
#93063=EDGE_LOOP ( 'NONE', ( #36689, #98498, #126950, #7092 ) ) ;
#93064=ORIENTED_EDGE ( 'NONE', *, *, #95361, .F. ) ;
#93066=DIRECTION ( 'NONE',  ( 0.000000000000000000, 1.000000000000000000, 0.000000000000000000 ) ) ;
#93067=EDGE_CURVE ( 'NONE', #34614, #59330, #10943, .T. ) ;
#93070=AXIS2_PLACEMENT_3D ( 'NONE', #32306, #51925, #11344 ) ;
#93071=VECTOR ( 'NONE', #80385, 1000.000000000000000 ) ;
#93072=AXIS2_PLACEMENT_3D ( 'NONE', #57728, #87161, #128415 ) ;
#93073=DIRECTION ( 'NONE',  ( -0.000000000000000000, 1.000000000000000000, -0.000000000000000000 ) ) ;
#93074=FACE_OUTER_BOUND ( 'NONE', #127313, .T. ) ;
#93075=PLANE ( 'NONE',  #122528 ) ;
#93076=DIRECTION ( 'NONE',  ( 0.000000000000000000, -0.9999939076577903929, 0.003490651415223739937 ) ) ;
#93077=AXIS2_PLACEMENT_3D ( 'NONE', #64479, #93306, #35048 ) ;
#93079=VERTEX_POINT ( 'NONE', #11377 ) ;
#93080=VERTEX_POINT ( 'NONE', #128613 ) ;
#93081=DIRECTION ( 'NONE',  ( 0.000000000000000000, -0.000000000000000000, 1.000000000000000000 ) ) ;
#93082=ORIENTED_EDGE ( 'NONE', *, *, #122758, .F. ) ;
#93083=DIRECTION ( 'NONE',  ( 0.000000000000000000, 0.000000000000000000, 1.000000000000000000 ) ) ;
#93084=DIRECTION ( 'NONE',  ( 0.000000000000000000, 1.000000000000000000, 0.000000000000000000 ) ) ;
#93085=CIRCLE ( 'NONE', #118104, 0.1000000000000002554 ) ;
#93086=CARTESIAN_POINT ( 'NONE',  ( -1.450000000000035039, 12.50000000000000000, -6.906693963081115051 ) ) ;
#93087=EDGE_LOOP ( 'NONE', ( #294, #119735 ) ) ;
#93088=VERTEX_POINT ( 'NONE', #70310 ) ;
#93089=FACE_BOUND ( 'NONE', #112690, .T. ) ;
#93090=EDGE_LOOP ( 'NONE', ( #75125, #71530, #104844, #123515 ) ) ;
#93091=CARTESIAN_POINT ( 'NONE',  ( -14.39999999999998614, 2.500000000000000000, -0.3464101615137760715 ) ) ;
#93092=FACE_OUTER_BOUND ( 'NONE', #53831, .T. ) ;
#93093=CARTESIAN_POINT ( 'NONE',  ( 3.549999999999943867, 2.500000000000000000, -6.148780366869526226 ) ) ;
#93094=CARTESIAN_POINT ( 'NONE',  ( 4.149999999999938183, 2.500000000000000000, 5.802370205355744659 ) ) ;
#93095=CARTESIAN_POINT ( 'NONE',  ( -2.900000000000029665, 2.500000000000000000, 3.637306695894644726 ) ) ;
#93096=CARTESIAN_POINT ( 'NONE',  ( 2.049999999999948308, 2.500000000000000000, 6.495190528383297135 ) ) ;
#93097=LINE ( 'NONE', #52505, #118775 ) ;
#93098=LINE ( 'NONE', #5336, #9807 ) ;
#93100=DIRECTION ( 'NONE',  ( -0.000000000000000000, 1.000000000000000000, -0.000000000000000000 ) ) ;
#93101=CIRCLE ( 'NONE', #105711, 0.06509327318403745899 ) ;
#93102=DIRECTION ( 'NONE',  ( 0.000000000000000000, 0.000000000000000000, -1.000000000000000000 ) ) ;
#93103=VERTEX_POINT ( 'NONE', #31051 ) ;
#93104=EDGE_LOOP ( 'NONE', ( #9928, #72291 ) ) ;
#93105=ADVANCED_FACE ( 'NONE', ( #119389 ), #128053, .T. ) ;
#93106=VERTEX_POINT ( 'NONE', #10095 ) ;
#93107=CARTESIAN_POINT ( 'NONE',  ( -7.700000000000016165, 2.500000000000000000, 0.3464101615137735735 ) ) ;
#93108=ORIENTED_EDGE ( 'NONE', *, *, #121071, .T. ) ;
#93109=DIRECTION ( 'NONE',  ( -0.000000000000000000, -1.000000000000000000, -0.000000000000000000 ) ) ;
#93110=VERTEX_POINT ( 'NONE', #38945 ) ;
#93111=ORIENTED_EDGE ( 'NONE', *, *, #96213, .T. ) ;
#93112=CONICAL_SURFACE ( 'NONE', #101512, 0.1000000000000000056, 0.003490658503988666988 ) ;
#93113=ORIENTED_EDGE ( 'NONE', *, *, #15863, .T. ) ;
#93114=CARTESIAN_POINT ( 'NONE',  ( 7.899999999999921307, 2.500000000000000000, -2.385244779468109755E-15 ) ) ;
#93115=AXIS2_PLACEMENT_3D ( 'NONE', #17220, #128531, #69570 ) ;
#93116=DIRECTION ( 'NONE',  ( -0.000000000000000000, 1.000000000000000000, -0.000000000000000000 ) ) ;
#93117=CARTESIAN_POINT ( 'NONE',  ( -0.8500000000000390576, 2.500000000000000000, -2.265063509461101798 ) ) ;
#93118=CARTESIAN_POINT ( 'NONE',  ( 26.76176526821260282, -1.073658814954678631, -4.445806700280396484 ) ) ;
#93119=LINE ( 'NONE', #101646, #93643 ) ;
#93120=CARTESIAN_POINT ( 'NONE',  ( 4.349999999999940137, 12.50000000000000000, -2.446380397790840266 ) ) ;
#93121=ADVANCED_FACE ( 'NONE', ( #110856 ), #50049, .T. ) ;
#93122=ORIENTED_EDGE ( 'NONE', *, *, #129499, .T. ) ;
#93123=DIRECTION ( 'NONE',  ( -0.000000000000000000, 1.000000000000000000, -0.000000000000000000 ) ) ;
#93124=ORIENTED_EDGE ( 'NONE', *, *, #36321, .T. ) ;
#93125=AXIS2_PLACEMENT_3D ( 'NONE', #23002, #93030, #74029 ) ;
#93126=ORIENTED_EDGE ( 'NONE', *, *, #29329, .F. ) ;
#93127=ORIENTED_EDGE ( 'NONE', *, *, #85616, .F. ) ;
#93128=VECTOR ( 'NONE', #126881, 1000.000000000000000 ) ;
#93129=DIRECTION ( 'NONE',  ( 0.000000000000000000, -0.000000000000000000, 1.000000000000000000 ) ) ;
#93130=ORIENTED_EDGE ( 'NONE', *, *, #80871, .F. ) ;
#93131=ORIENTED_EDGE ( 'NONE', *, *, #120396, .T. ) ;
#93132=EDGE_LOOP ( 'NONE', ( #93991, #34712, #39591, #38063 ) ) ;
#93133=FACE_OUTER_BOUND ( 'NONE', #63920, .T. ) ;
#93134=DIRECTION ( 'NONE',  ( 0.000000000000000000, 1.000000000000000000, 0.000000000000000000 ) ) ;
#93135=AXIS2_PLACEMENT_3D ( 'NONE', #76153, #116706, #54555 ) ;
#93136=CARTESIAN_POINT ( 'NONE',  ( 10.84999999999991260, 12.50000000000000000, -1.472243186433550122 ) ) ;
#93137=DIRECTION ( 'NONE',  ( 0.000000000000000000, -0.9999939076577903929, 0.003490651415223739937 ) ) ;
#93138=DIRECTION ( 'NONE',  ( -0.000000000000000000, -1.000000000000000000, -0.000000000000000000 ) ) ;
#93139=DIRECTION ( 'NONE',  ( 0.000000000000000000, 0.000000000000000000, -1.000000000000000000 ) ) ;
#93140=FACE_OUTER_BOUND ( 'NONE', #41418, .T. ) ;
#93141=VERTEX_POINT ( 'NONE', #69005 ) ;
#93142=DIRECTION ( 'NONE',  ( -0.000000000000000000, -1.000000000000000000, -0.000000000000000000 ) ) ;
#93143=EDGE_CURVE ( 'NONE', #33550, #38354, #100843, .T. ) ;
#93144=ORIENTED_EDGE ( 'NONE', *, *, #115878, .F. ) ;
#93145=DIRECTION ( 'NONE',  ( 0.000000000000000000, 1.000000000000000000, 0.000000000000000000 ) ) ;
#93146=AXIS2_PLACEMENT_3D ( 'NONE', #81024, #20167, #49647 ) ;
#93147=ORIENTED_EDGE ( 'NONE', *, *, #83808, .F. ) ;
#93148=CIRCLE ( 'NONE', #13700, 0.09999999999999982514 ) ;
#93149=EDGE_LOOP ( 'NONE', ( #7062, #65351 ) ) ;
#93150=EDGE_CURVE ( 'NONE', #121438, #77033, #40224, .T. ) ;
#93151=DIRECTION ( 'NONE',  ( 0.000000000000000000, -0.000000000000000000, 1.000000000000000000 ) ) ;
#93152=FACE_OUTER_BOUND ( 'NONE', #82799, .T. ) ;
#93153=CIRCLE ( 'NONE', #82695, 0.06509327318403745899 ) ;
#93154=VECTOR ( 'NONE', #110844, 1000.000000000000000 ) ;
#93155=DIRECTION ( 'NONE',  ( -4.274815082592931898E-19, -0.9999939076577903929, -0.003490651415223739937 ) ) ;
#93156=ORIENTED_EDGE ( 'NONE', *, *, #45590, .F. ) ;
#93157=ADVANCED_FACE ( 'NONE', ( #30407 ), #80785, .T. ) ;
#93158=EDGE_CURVE ( 'NONE', #92121, #40225, #46468, .T. ) ;
#93159=ORIENTED_EDGE ( 'NONE', *, *, #92729, .F. ) ;
#93160=DIRECTION ( 'NONE',  ( -0.000000000000000000, 1.000000000000000000, -0.000000000000000000 ) ) ;
#93161=DIRECTION ( 'NONE',  ( 0.000000000000000000, 0.000000000000000000, 1.000000000000000000 ) ) ;
#93162=EDGE_CURVE ( 'NONE', #82670, #107304, #19251, .T. ) ;
#93163=CARTESIAN_POINT ( 'NONE',  ( 2.099999999999950351, 12.50000000000000000, -4.395220292106239768 ) ) ;
#93164=EDGE_CURVE ( 'NONE', #63587, #120581, #6732, .T. ) ;
#93165=EDGE_CURVE ( 'NONE', #120897, #27524, #4761, .T. ) ;
#93166=DIRECTION ( 'NONE',  ( 0.000000000000000000, -0.000000000000000000, 1.000000000000000000 ) ) ;
#93167=CIRCLE ( 'NONE', #9530, 0.1000000000000002554 ) ;
#93168=LINE ( 'NONE', #101689, #112758 ) ;
#93169=ORIENTED_EDGE ( 'NONE', *, *, #104227, .F. ) ;
#93170=CARTESIAN_POINT ( 'NONE',  ( -13.29999999999998828, 2.500000000000000000, 4.330127018922196314 ) ) ;
#93171=EDGE_CURVE ( 'NONE', #114482, #85021, #44422, .T. ) ;
#93172=ORIENTED_EDGE ( 'NONE', *, *, #95198, .F. ) ;
#93173=EDGE_CURVE ( 'NONE', #1061, #37867, #61791, .T. ) ;
#93174=CIRCLE ( 'NONE', #114089, 0.06509327318403745899 ) ;
#93175=PLANE ( 'NONE',  #8916 ) ;
#93176=CARTESIAN_POINT ( 'NONE',  ( 10.19999999999991047, 12.50000000000000000, -3.918623584224389056 ) ) ;
#93177=AXIS2_PLACEMENT_3D ( 'NONE', #828, #28369, #118663 ) ;
#93178=EDGE_CURVE ( 'NONE', #93002, #83416, #109357, .T. ) ;
#93179=AXIS2_PLACEMENT_3D ( 'NONE', #42081, #40145, #40809 ) ;
#93180=VECTOR ( 'NONE', #87174, 1000.000000000000000 ) ;
#93182=FACE_OUTER_BOUND ( 'NONE', #123353, .T. ) ;
#93183=DIRECTION ( 'NONE',  ( 0.000000000000000000, -0.000000000000000000, 1.000000000000000000 ) ) ;
#93184=CARTESIAN_POINT ( 'NONE',  ( -3.950000000000025491, 2.500000000000000000, 6.148780366869520897 ) ) ;
#93185=CARTESIAN_POINT ( 'NONE',  ( -6.450000000000014388, 2.500000000000000000, 6.148780366869520897 ) ) ;
#93187=DIRECTION ( 'NONE',  ( 0.000000000000000000, 0.000000000000000000, 1.000000000000000000 ) ) ;
#93188=DIRECTION ( 'NONE',  ( -0.000000000000000000, -1.000000000000000000, -0.000000000000000000 ) ) ;
#93189=DIRECTION ( 'NONE',  ( 0.000000000000000000, 0.000000000000000000, -1.000000000000000000 ) ) ;
#93190=VERTEX_POINT ( 'NONE', #111510 ) ;
#93191=CIRCLE ( 'NONE', #80667, 0.1000000000000002554 ) ;
#93192=DIRECTION ( 'NONE',  ( -0.000000000000000000, 1.000000000000000000, -0.000000000000000000 ) ) ;
#93193=EDGE_LOOP ( 'NONE', ( #106308, #30428, #28553, #84502 ) ) ;
#93194=DIRECTION ( 'NONE',  ( 0.000000000000000000, 1.000000000000000000, 0.000000000000000000 ) ) ;
#93195=AXIS2_PLACEMENT_3D ( 'NONE', #66815, #6585, #106746 ) ;
#93196=ORIENTED_EDGE ( 'NONE', *, *, #119233, .F. ) ;
#93197=CARTESIAN_POINT ( 'NONE',  ( 19.08853762628606532, -0.5565172523996277931, -4.470057054644892780 ) ) ;
#93198=DIRECTION ( 'NONE',  ( -4.274815082592931898E-19, -0.9999939076577903929, -0.003490651415223739937 ) ) ;
#93199=CARTESIAN_POINT ( 'NONE',  ( -14.39999999999998614, 2.500000000000000000, 0.2464101615137758439 ) ) ;
#93200=CIRCLE ( 'NONE', #9572, 0.06509327318403745899 ) ;
#93201=ORIENTED_EDGE ( 'NONE', *, *, #23119, .T. ) ;
#93202=DIRECTION ( 'NONE',  ( 0.000000000000000000, 1.000000000000000000, 0.000000000000000000 ) ) ;
#93203=CIRCLE ( 'NONE', #43139, 0.06509327318403745899 ) ;
#93204=CARTESIAN_POINT ( 'NONE',  ( -11.64999999999999680, 2.500000000000000000, 2.757883832488649656 ) ) ;
#93205=ADVANCED_FACE ( 'NONE', ( #33608 ), #36214, .T. ) ;
#93206=EDGE_LOOP ( 'NONE', ( #41694, #87784 ) ) ;
#93207=ADVANCED_FACE ( 'NONE', ( #112813 ), #29853, .T. ) ;
#93208=ORIENTED_EDGE ( 'NONE', *, *, #12618, .T. ) ;
#93209=AXIS2_PLACEMENT_3D ( 'NONE', #45138, #77166, #35320 ) ;
#93210=CIRCLE ( 'NONE', #89099, 0.06509327318403745899 ) ;
#93211=EDGE_CURVE ( 'NONE', #109920, #5141, #54514, .T. ) ;
#93212=VERTEX_POINT ( 'NONE', #44722 ) ;
#93213=DIRECTION ( 'NONE',  ( -0.000000000000000000, -1.000000000000000000, -0.000000000000000000 ) ) ;
#93214=DIRECTION ( 'NONE',  ( 0.000000000000000000, 0.000000000000000000, 1.000000000000000000 ) ) ;
#93215=CARTESIAN_POINT ( 'NONE',  ( 11.64999999999990266, 2.500000000000000000, 2.165063509461097713 ) ) ;
#93216=ORIENTED_EDGE ( 'NONE', *, *, #106313, .F. ) ;
#93217=DIRECTION ( 'NONE',  ( 0.000000000000000000, 0.000000000000000000, 1.000000000000000000 ) ) ;
#93218=DIRECTION ( 'NONE',  ( 0.000000000000000000, -0.000000000000000000, 1.000000000000000000 ) ) ;
#93219=ORIENTED_EDGE ( 'NONE', *, *, #24547, .F. ) ;
#93220=ADVANCED_FACE ( 'NONE', ( #13949 ), #92634, .T. ) ;
#93221=FACE_OUTER_BOUND ( 'NONE', #110034, .T. ) ;
#93222=VECTOR ( 'NONE', #50539, 1000.000000000000000 ) ;
#93223=FACE_OUTER_BOUND ( 'NONE', #60522, .T. ) ;
#93224=DIRECTION ( 'NONE',  ( 0.000000000000000000, 1.000000000000000000, 0.000000000000000000 ) ) ;
#93225=PLANE ( 'NONE',  #111981 ) ;
#93226=DIRECTION ( 'NONE',  ( 0.000000000000000000, -0.9999939076577903929, 0.003490651415223739937 ) ) ;
#93227=FACE_OUTER_BOUND ( 'NONE', #100116, .T. ) ;
#93228=CARTESIAN_POINT ( 'NONE',  ( -5.850000000000021849, 12.50000000000000000, -7.253104124594891289 ) ) ;
#93230=VERTEX_POINT ( 'NONE', #123906 ) ;
#93231=ORIENTED_EDGE ( 'NONE', *, *, #62156, .F. ) ;
#93232=EDGE_LOOP ( 'NONE', ( #59606, #53568, #81620, #50969 ) ) ;
#93233=CARTESIAN_POINT ( 'NONE',  ( 48.81612456492386087, 3.619496399135581743, 4.312668942933988170 ) ) ;
#93234=DIRECTION ( 'NONE',  ( -0.000000000000000000, 1.000000000000000000, -0.000000000000000000 ) ) ;
#93235=DIRECTION ( 'NONE',  ( 0.000000000000000000, 0.000000000000000000, -1.000000000000000000 ) ) ;
#93236=ORIENTED_EDGE ( 'NONE', *, *, #17664, .F. ) ;
#93237=FACE_BOUND ( 'NONE', #98708, .T. ) ;
#93238=ADVANCED_FACE ( 'NONE', ( #103639 ), #71592, .T. ) ;
#93239=DIRECTION ( 'NONE',  ( 0.000000000000000000, 1.000000000000000000, 0.000000000000000000 ) ) ;
#93240=DIRECTION ( 'NONE',  ( -0.000000000000000000, -1.000000000000000000, -0.000000000000000000 ) ) ;
#93241=DIRECTION ( 'NONE',  ( -0.000000000000000000, 1.000000000000000000, -0.000000000000000000 ) ) ;
#93242=CONICAL_SURFACE ( 'NONE', #89119, 0.1000000000000002554, 0.003490658503988666988 ) ;
#93243=FACE_OUTER_BOUND ( 'NONE', #99418, .T. ) ;
#93244=AXIS2_PLACEMENT_3D ( 'NONE', #12493, #91708, #52419 ) ;
#93245=DIRECTION ( 'NONE',  ( 0.000000000000000000, 1.000000000000000000, 0.000000000000000000 ) ) ;
#93246=CARTESIAN_POINT ( 'NONE',  ( -6.850000000000017408, 12.50000000000000000, -1.818653347947325916 ) ) ;
#93247=DIRECTION ( 'NONE',  ( 0.000000000000000000, -0.9999939076577903929, 0.003490651415223739937 ) ) ;
#93248=CARTESIAN_POINT ( 'NONE',  ( 3.949999999999941558, 2.500000000000000000, -6.148780366869526226 ) ) ;
#93249=DIRECTION ( 'NONE',  ( 0.000000000000000000, 0.000000000000000000, 1.000000000000000000 ) ) ;
#93250=CONICAL_SURFACE ( 'NONE', #7547, 0.09999999999999999167, 0.003490658503988666988 ) ;
#93251=ORIENTED_EDGE ( 'NONE', *, *, #12258, .F. ) ;
#93252=ORIENTED_EDGE ( 'NONE', *, *, #26216, .F. ) ;
#93253=ORIENTED_EDGE ( 'NONE', *, *, #89737, .F. ) ;
#93254=EDGE_CURVE ( 'NONE', #96534, #61265, #82173, .T. ) ;
#93255=ORIENTED_EDGE ( 'NONE', *, *, #99926, .F. ) ;
#93257=ORIENTED_EDGE ( 'NONE', *, *, #31938, .T. ) ;
#93258=CARTESIAN_POINT ( 'NONE',  ( -1.050000000000038236, 2.500000000000000000, -1.818653347947326138 ) ) ;
#93259=VERTEX_POINT ( 'NONE', #43443 ) ;
#93260=EDGE_LOOP ( 'NONE', ( #70485, #119790, #103822, #77754 ) ) ;
#93261=AXIS2_PLACEMENT_3D ( 'NONE', #58396, #116645, #16499 ) ;
#93262=AXIS2_PLACEMENT_3D ( 'NONE', #67479, #117885, #26946 ) ;
#93263=CARTESIAN_POINT ( 'NONE',  ( 0.1999999999999571565, 2.500000000000000000, 3.983716857408420076 ) ) ;
#93264=CARTESIAN_POINT ( 'NONE',  ( 7.699999999999923794, 12.50000000000000000, 4.676537180435972552 ) ) ;
#93265=DIRECTION ( 'NONE',  ( -4.274815082592931898E-19, -0.9999939076577903929, -0.003490651415223739937 ) ) ;
#93266=EDGE_CURVE ( 'NONE', #56139, #116013, #128146, .T. ) ;
#93267=ORIENTED_EDGE ( 'NONE', *, *, #80197, .F. ) ;
#93268=CARTESIAN_POINT ( 'NONE',  ( 6.649999999999931077, 12.50000000000000000, -6.495190528383302464 ) ) ;
#93269=ORIENTED_EDGE ( 'NONE', *, *, #77237, .F. ) ;
#93270=ORIENTED_EDGE ( 'NONE', *, *, #86803, .T. ) ;
#93271=FACE_OUTER_BOUND ( 'NONE', #81671, .T. ) ;
#93272=FACE_OUTER_BOUND ( 'NONE', #91854, .T. ) ;
#93273=AXIS2_PLACEMENT_3D ( 'NONE', #15624, #125581, #56827 ) ;
#93274=ORIENTED_EDGE ( 'NONE', *, *, #93006, .F. ) ;
#93275=VERTEX_POINT ( 'NONE', #114096 ) ;
#93276=CARTESIAN_POINT ( 'NONE',  ( -6.850000000000017408, 2.500000000000000000, -6.841600689897077814 ) ) ;
#93277=LINE ( 'NONE', #73619, #106002 ) ;
#93279=DIRECTION ( 'NONE',  ( 0.000000000000000000, -0.9999939076577903929, 0.003490651415223739937 ) ) ;
#93280=DIRECTION ( 'NONE',  ( 0.000000000000000000, 0.000000000000000000, 1.000000000000000000 ) ) ;
#93281=CONICAL_SURFACE ( 'NONE', #24320, 0.1000000000000002554, 0.003490658503988666988 ) ;
#93282=CIRCLE ( 'NONE', #84955, 0.06509327318403741736 ) ;
#93283=ORIENTED_EDGE ( 'NONE', *, *, #119233, .T. ) ;
#93284=DIRECTION ( 'NONE',  ( 0.000000000000000000, 0.000000000000000000, 1.000000000000000000 ) ) ;
#93285=VERTEX_POINT ( 'NONE', #42137 ) ;
#93286=CARTESIAN_POINT ( 'NONE',  ( 87.50000000000002842, 7.500000000000000888, 0.6928095518838445210 ) ) ;
#93287=ADVANCED_FACE ( 'NONE', ( #121987 ), #102352, .T. ) ;
#93288=ORIENTED_EDGE ( 'NONE', *, *, #52052, .T. ) ;
#93289=DIRECTION ( 'NONE',  ( 0.000000000000000000, 1.000000000000000000, 0.000000000000000000 ) ) ;
#93290=CARTESIAN_POINT ( 'NONE',  ( 11.89999999999990443, 2.500000000000000000, 0.2464101615137736789 ) ) ;
#93291=LINE ( 'NONE', #49683, #115528 ) ;
#93292=DIRECTION ( 'NONE',  ( -4.274815082592931898E-19, -0.9999939076577903929, -0.003490651415223739937 ) ) ;
#93293=ORIENTED_EDGE ( 'NONE', *, *, #95342, .T. ) ;
#93294=AXIS2_PLACEMENT_3D ( 'NONE', #69861, #50231, #8987 ) ;
#93295=EDGE_CURVE ( 'NONE', #93509, #80466, #52834, .T. ) ;
#93296=CARTESIAN_POINT ( 'NONE',  ( -1.650000000000034328, 2.500000000000000000, -2.857883832488653741 ) ) ;
#93297=CIRCLE ( 'NONE', #99573, 0.09999999999999982514 ) ;
#93298=AXIS2_PLACEMENT_3D ( 'NONE', #72006, #91631, #33379 ) ;
#93299=DIRECTION ( 'NONE',  ( -0.000000000000000000, -1.000000000000000000, -0.000000000000000000 ) ) ;
#93300=ORIENTED_EDGE ( 'NONE', *, *, #1652, .F. ) ;
#93301=ORIENTED_EDGE ( 'NONE', *, *, #46638, .F. ) ;
#93302=ADVANCED_FACE ( 'NONE', ( #63062 ), #25726, .T. ) ;
#93303=EDGE_CURVE ( 'NONE', #3765, #43648, #117645, .T. ) ;
#93304=ORIENTED_EDGE ( 'NONE', *, *, #53036, .T. ) ;
#93305=FACE_OUTER_BOUND ( 'NONE', #61747, .T. ) ;
#93306=DIRECTION ( 'NONE',  ( 0.000000000000000000, 1.000000000000000000, 0.000000000000000000 ) ) ;
#93307=EDGE_CURVE ( 'NONE', #31124, #120269, #122631, .T. ) ;
#93309=ADVANCED_FACE ( 'NONE', ( #56451 ), #46011, .T. ) ;
#93310=DIRECTION ( 'NONE',  ( 0.000000000000000000, 0.000000000000000000, -1.000000000000000000 ) ) ;
#93311=DIRECTION ( 'NONE',  ( 0.000000000000000000, 0.000000000000000000, 1.000000000000000000 ) ) ;
#93312=FACE_OUTER_BOUND ( 'NONE', #38913, .T. ) ;
#93313=DIRECTION ( 'NONE',  ( 0.000000000000000000, -0.9999939076577903929, 0.003490651415223739937 ) ) ;
#93314=EDGE_CURVE ( 'NONE', #43343, #109816, #95747, .T. ) ;
#93315=EDGE_CURVE ( 'NONE', #15536, #105793, #57023, .T. ) ;
#93316=ADVANCED_FACE ( 'NONE', ( #79182 ), #25068, .T. ) ;
#93317=ORIENTED_EDGE ( 'NONE', *, *, #17151, .T. ) ;
#93318=EDGE_CURVE ( 'NONE', #21011, #54541, #65436, .T. ) ;
#93319=DIRECTION ( 'NONE',  ( 0.000000000000000000, 1.000000000000000000, 0.000000000000000000 ) ) ;
#93320=EDGE_CURVE ( 'NONE', #68464, #16720, #102997, .T. ) ;
#93321=VERTEX_POINT ( 'NONE', #125834 ) ;
#93322=LINE ( 'NONE', #125822, #94512 ) ;
#93323=DIRECTION ( 'NONE',  ( 0.000000000000000000, 1.000000000000000000, 0.000000000000000000 ) ) ;
#93324=DIRECTION ( 'NONE',  ( 0.000000000000000000, 0.000000000000000000, 1.000000000000000000 ) ) ;
#93325=DIRECTION ( 'NONE',  ( 0.000000000000000000, 0.000000000000000000, 1.000000000000000000 ) ) ;
#93326=EDGE_CURVE ( 'NONE', #102605, #88147, #119722, .T. ) ;
#93327=EDGE_LOOP ( 'NONE', ( #35097, #127653, #127423, #50148 ) ) ;
#93328=CIRCLE ( 'NONE', #11834, 0.06509327318403745899 ) ;
#93329=AXIS2_PLACEMENT_3D ( 'NONE', #65453, #43271, #114553 ) ;
#93330=PLANE ( 'NONE',  #15775 ) ;
#93331=CARTESIAN_POINT ( 'NONE',  ( 4.549999999999935874, 2.500000000000000000, 6.495190528383297135 ) ) ;
#93332=VERTEX_POINT ( 'NONE', #114732 ) ;
#93333=EDGE_LOOP ( 'NONE', ( #65403, #84586 ) ) ;
#93334=CIRCLE ( 'NONE', #36911, 0.06509327318403743123 ) ;
#93335=AXIS2_PLACEMENT_3D ( 'NONE', #82275, #23993, #22717 ) ;
#93336=CARTESIAN_POINT ( 'NONE',  ( -11.89999999999999503, 2.500000000000000000, 3.983716857408420076 ) ) ;
#93337=EDGE_LOOP ( 'NONE', ( #111460, #51447, #47617, #53186 ) ) ;
#93338=VERTEX_POINT ( 'NONE', #29429 ) ;
#93339=CARTESIAN_POINT ( 'NONE',  ( -7.100000000000018296, 12.50000000000000000, 0.06509327318403504425 ) ) ;
#93340=VERTEX_POINT ( 'NONE', #6682 ) ;
#93341=CARTESIAN_POINT ( 'NONE',  ( 16.86689433361523172, 2.548103353433960994, -5.776876940644999792 ) ) ;
#93342=DIRECTION ( 'NONE',  ( -4.274815082592931898E-19, -0.9999939076577903929, -0.003490651415223739937 ) ) ;
#93343=VECTOR ( 'NONE', #89126, 1000.000000000000000 ) ;
#93344=CIRCLE ( 'NONE', #124656, 0.06509327318403745899 ) ;
#93345=CARTESIAN_POINT ( 'NONE',  ( -2.500000000000030642, 12.50000000000000000, -5.022947341949754119 ) ) ;
#93346=ORIENTED_EDGE ( 'NONE', *, *, #93721, .F. ) ;
#93347=CONICAL_SURFACE ( 'NONE', #57855, 0.09999999999999982514, 0.003490658503988666988 ) ;
#93348=FACE_OUTER_BOUND ( 'NONE', #39612, .T. ) ;
#93349=CARTESIAN_POINT ( 'NONE',  ( -6.700000000000016165, 12.50000000000000000, 4.330127018922196314 ) ) ;
#93350=EDGE_LOOP ( 'NONE', ( #141, #99744 ) ) ;
#93351=CARTESIAN_POINT ( 'NONE',  ( 17.50011901588676722, 2.224285231026832843, 4.071013062215452116 ) ) ;
#93352=LINE ( 'NONE', #22048, #38372 ) ;
#93353=ORIENTED_EDGE ( 'NONE', *, *, #21344, .F. ) ;
#93354=ADVANCED_FACE ( 'NONE', ( #9776 ), #63295, .T. ) ;
#93355=EDGE_LOOP ( 'NONE', ( #44075, #118929, #44361, #119843 ) ) ;
#93356=EDGE_CURVE ( 'NONE', #99398, #54553, #125206, .T. ) ;
#93357=ORIENTED_EDGE ( 'NONE', *, *, #102720, .T. ) ;
#93358=EDGE_LOOP ( 'NONE', ( #8379, #8907 ) ) ;
#93359=DIRECTION ( 'NONE',  ( 0.000000000000000000, -0.9999939076577903929, 0.003490651415223739937 ) ) ;
#93360=CARTESIAN_POINT ( 'NONE',  ( -2.100000000000033396, 2.500000000000000000, 0.6928203230275494784 ) ) ;
#93361=DIRECTION ( 'NONE',  ( -0.000000000000000000, 1.000000000000000000, -0.000000000000000000 ) ) ;
#93362=FACE_BOUND ( 'NONE', #22133, .T. ) ;
#93363=VERTEX_POINT ( 'NONE', #57103 ) ;
#93364=AXIS2_PLACEMENT_3D ( 'NONE', #113698, #63299, #51563 ) ;
#93366=DIRECTION ( 'NONE',  ( 0.000000000000000000, -0.9999939076577903929, 0.003490651415223739937 ) ) ;
#93367=DIRECTION ( 'NONE',  ( -0.000000000000000000, 1.000000000000000000, -0.000000000000000000 ) ) ;
#93368=CIRCLE ( 'NONE', #104115, 0.06509327318403745899 ) ;
#93369=EDGE_CURVE ( 'NONE', #94125, #52738, #6830, .T. ) ;
#93370=AXIS2_PLACEMENT_3D ( 'NONE', #77558, #17996, #78232 ) ;
#93372=CARTESIAN_POINT ( 'NONE',  ( -8.350000000000013856, 2.500000000000000000, -7.188010851410848723 ) ) ;
#93373=CARTESIAN_POINT ( 'NONE',  ( -5.400000000000020783, 2.500000000000000000, 4.922947341949748257 ) ) ;
#93374=AXIS2_PLACEMENT_3D ( 'NONE', #73732, #113678, #74392 ) ;
#93375=CONICAL_SURFACE ( 'NONE', #35003, 0.1000000000000002554, 0.003490658503988666988 ) ;
#93376=LINE ( 'NONE', #122834, #80824 ) ;
#93377=AXIS2_PLACEMENT_3D ( 'NONE', #47030, #45096, #84994 ) ;
#93378=ORIENTED_EDGE ( 'NONE', *, *, #111801, .T. ) ;
#93379=EDGE_LOOP ( 'NONE', ( #106596, #65658 ) ) ;
#93380=EDGE_LOOP ( 'NONE', ( #88714, #40448 ) ) ;
#93381=EDGE_LOOP ( 'NONE', ( #1743, #102524 ) ) ;
#93382=ORIENTED_EDGE ( 'NONE', *, *, #60426, .T. ) ;
#93383=DIRECTION ( 'NONE',  ( -0.000000000000000000, 1.000000000000000000, -0.000000000000000000 ) ) ;
#93384=DIRECTION ( 'NONE',  ( 0.000000000000000000, 1.000000000000000000, 0.000000000000000000 ) ) ;
#93385=CONICAL_SURFACE ( 'NONE', #39126, 0.09999999999999982514, 0.003490658503988666988 ) ;
#93386=EDGE_LOOP ( 'NONE', ( #48571, #129467 ) ) ;
#93387=FACE_BOUND ( 'NONE', #29272, .T. ) ;
#93388=AXIS2_PLACEMENT_3D ( 'NONE', #14611, #25096, #61331 ) ;
#93389=CARTESIAN_POINT ( 'NONE',  ( -10.85000000000000142, 12.50000000000000000, 6.495190528383297135 ) ) ;
#93390=CONICAL_SURFACE ( 'NONE', #105910, 0.09999999999999999167, 0.003490658503988666988 ) ;
#93391=CIRCLE ( 'NONE', #36963, 0.06509327318403745899 ) ;
#93392=VERTEX_POINT ( 'NONE', #76105 ) ;
#93393=CARTESIAN_POINT ( 'NONE',  ( 10.84999999999990905, 12.50000000000000000, -7.188010851410854052 ) ) ;
#93394=DIRECTION ( 'NONE',  ( 0.000000000000000000, 0.000000000000000000, -1.000000000000000000 ) ) ;
#93395=CARTESIAN_POINT ( 'NONE',  ( 7.899999999999924860, 12.50000000000000000, 5.088040615133786027 ) ) ;
#93396=VERTEX_POINT ( 'NONE', #65631 ) ;
#93397=DIRECTION ( 'NONE',  ( 0.000000000000000000, 0.000000000000000000, 1.000000000000000000 ) ) ;
#93398=ADVANCED_FACE ( 'NONE', ( #34913 ), #128938, .T. ) ;
#93399=ORIENTED_EDGE ( 'NONE', *, *, #81181, .T. ) ;
#93400=ORIENTED_EDGE ( 'NONE', *, *, #108092, .T. ) ;
#93401=EDGE_LOOP ( 'NONE', ( #128181, #63812 ) ) ;
#93402=FACE_OUTER_BOUND ( 'NONE', #44763, .T. ) ;
#93403=CARTESIAN_POINT ( 'NONE',  ( 11.69999999999990514, 2.500000000000000000, -2.276824562219559311E-15 ) ) ;
#93404=PLANE ( 'NONE',  #38392 ) ;
#93405=ORIENTED_EDGE ( 'NONE', *, *, #2053, .T. ) ;
#93406=AXIS2_PLACEMENT_3D ( 'NONE', #33224, #14819, #43054 ) ;
#93407=DIRECTION ( 'NONE',  ( 0.000000000000000000, 0.000000000000000000, 1.000000000000000000 ) ) ;
#93408=CARTESIAN_POINT ( 'NONE',  ( -14.14999999999998614, 12.50000000000000000, -2.857883832488651521 ) ) ;
#93409=FACE_OUTER_BOUND ( 'NONE', #41839, .T. ) ;
#93411=ORIENTED_EDGE ( 'NONE', *, *, #88908, .T. ) ;
#93412=ADVANCED_FACE ( 'NONE', ( #96367 ), #42478, .T. ) ;
#93413=DIRECTION ( 'NONE',  ( 0.000000000000000000, 1.000000000000000000, 0.000000000000000000 ) ) ;
#93414=EDGE_CURVE ( 'NONE', #97521, #2455, #54974, .T. ) ;
#93415=ORIENTED_EDGE ( 'NONE', *, *, #97695, .T. ) ;
#93416=DIRECTION ( 'NONE',  ( 0.000000000000000000, -0.000000000000000000, 1.000000000000000000 ) ) ;
#93417=CIRCLE ( 'NONE', #13974, 0.06509327318403745899 ) ;
#93418=ORIENTED_EDGE ( 'NONE', *, *, #70009, .F. ) ;
#93419=AXIS2_PLACEMENT_3D ( 'NONE', #40544, #80458, #90907 ) ;
#93420=ORIENTED_EDGE ( 'NONE', *, *, #114450, .T. ) ;
#93421=DIRECTION ( 'NONE',  ( -4.274815082592931898E-19, -0.9999939076577903929, -0.003490651415223739937 ) ) ;
#93422=PLANE ( 'NONE',  #25697 ) ;
#93423=CARTESIAN_POINT ( 'NONE',  ( -5.600000000000020073, 2.500000000000000000, -0.3464101615137782364 ) ) ;
#93424=PLANE ( 'NONE',  #69626 ) ;
#93425=ADVANCED_FACE ( 'NONE', ( #66280 ), #588, .T. ) ;
#93426=DIRECTION ( 'NONE',  ( -4.274815082592931898E-19, -0.9999939076577903929, -0.003490651415223739937 ) ) ;
#93427=ORIENTED_EDGE ( 'NONE', *, *, #128621, .F. ) ;
#93428=AXIS2_PLACEMENT_3D ( 'NONE', #1256, #18941, #11714 ) ;
#93429=AXIS2_PLACEMENT_3D ( 'NONE', #94647, #3068, #84834 ) ;
#93430=EDGE_LOOP ( 'NONE', ( #62819, #57588 ) ) ;
#93431=DIRECTION ( 'NONE',  ( 0.000000000000000000, 1.000000000000000000, 0.000000000000000000 ) ) ;
#93432=CARTESIAN_POINT ( 'NONE',  ( -0.4000000000000392131, 2.500000000000000000, -4.330127018922201643 ) ) ;
#93433=DIRECTION ( 'NONE',  ( -0.000000000000000000, 1.000000000000000000, -0.000000000000000000 ) ) ;
#93434=ORIENTED_EDGE ( 'NONE', *, *, #96693, .F. ) ;
#93435=VERTEX_POINT ( 'NONE', #7346 ) ;
#93437=CONICAL_SURFACE ( 'NONE', #120628, 0.1000000000000000472, 0.003490658503988666988 ) ;
#93438=ORIENTED_EDGE ( 'NONE', *, *, #115019, .F. ) ;
#93439=DIRECTION ( 'NONE',  ( 0.000000000000000000, 1.000000000000000000, 0.000000000000000000 ) ) ;
#93440=DIRECTION ( 'NONE',  ( 0.000000000000000000, 0.000000000000000000, 1.000000000000000000 ) ) ;
#93441=VERTEX_POINT ( 'NONE', #88986 ) ;
#93442=CARTESIAN_POINT ( 'NONE',  ( 9.599999999999917932, 2.500000000000000000, -2.276824562219559311E-15 ) ) ;
#93443=CARTESIAN_POINT ( 'NONE',  ( -0.6000000000000388356, 2.500000000000000000, 3.883716857408421319 ) ) ;
#93444=DIRECTION ( 'NONE',  ( -4.274815082592931898E-19, -0.9999939076577903929, -0.003490651415223739937 ) ) ;
#93445=DIRECTION ( 'NONE',  ( -4.274815082592931898E-19, -0.9999939076577903929, -0.003490651415223739937 ) ) ;
#93446=VERTEX_POINT ( 'NONE', #39274 ) ;
#93448=DIRECTION ( 'NONE',  ( -0.000000000000000000, -1.000000000000000000, -0.000000000000000000 ) ) ;
#93449=CARTESIAN_POINT ( 'NONE',  ( 81.97673105525203141, -3.779183761609747005, 6.223416311177524918 ) ) ;
#93450=EDGE_LOOP ( 'NONE', ( #102738, #107970, #101327, #106691 ) ) ;
#93451=ORIENTED_EDGE ( 'NONE', *, *, #5394, .T. ) ;
#93452=ADVANCED_FACE ( 'NONE', ( #30086 ), #90466, .T. ) ;
#93454=FACE_OUTER_BOUND ( 'NONE', #44587, .T. ) ;
#93455=CONICAL_SURFACE ( 'NONE', #110187, 0.09999999999999982514, 0.003490658503988666988 ) ;
#93456=CARTESIAN_POINT ( 'NONE',  ( -2.050000000000032685, 12.50000000000000000, -6.430097255199264339 ) ) ;
#93457=AXIS2_PLACEMENT_3D ( 'NONE', #40634, #68769, #39970 ) ;
#93458=EDGE_CURVE ( 'NONE', #17249, #75945, #121874, .T. ) ;
#93459=CARTESIAN_POINT ( 'NONE',  ( 11.64999999999990621, 2.500000000000000000, -2.165063509461101710 ) ) ;
#93460=CIRCLE ( 'NONE', #28716, 0.06509327318403745899 ) ;
#93461=DIRECTION ( 'NONE',  ( 0.000000000000000000, 0.000000000000000000, -1.000000000000000000 ) ) ;
#93462=DIRECTION ( 'NONE',  ( -0.000000000000000000, -1.000000000000000000, -0.000000000000000000 ) ) ;
#93463=VECTOR ( 'NONE', #31073, 1000.000000000000000 ) ;
#93464=CARTESIAN_POINT ( 'NONE',  ( -8.749999999999971578, 2.500000000000000000, 6.395190528383296602 ) ) ;
#93465=CARTESIAN_POINT ( 'NONE',  ( -5.850000000000018296, 2.500000000000000000, 5.802370205355744659 ) ) ;
#93466=CARTESIAN_POINT ( 'NONE',  ( 3.549999999999942979, 2.500000000000000000, 1.918653347947321564 ) ) ;
#93467=DIRECTION ( 'NONE',  ( 0.000000000000000000, 0.000000000000000000, 1.000000000000000000 ) ) ;
#93468=EDGE_CURVE ( 'NONE', #115231, #122569, #4784, .T. ) ;
#93469=EDGE_CURVE ( 'NONE', #20166, #39360, #98890, .T. ) ;
#93471=AXIS2_PLACEMENT_3D ( 'NONE', #80205, #21265, #31746 ) ;
#93472=AXIS2_PLACEMENT_3D ( 'NONE', #56663, #106429, #54737 ) ;
#93473=CARTESIAN_POINT ( 'NONE',  ( -11.44999999999999751, 12.50000000000000000, 1.818653347947321475 ) ) ;
#93474=ORIENTED_EDGE ( 'NONE', *, *, #21663, .F. ) ;
#93475=ORIENTED_EDGE ( 'NONE', *, *, #86906, .F. ) ;
#93476=AXIS2_PLACEMENT_3D ( 'NONE', #76749, #37485, #48584 ) ;
#93477=EDGE_CURVE ( 'NONE', #119959, #63523, #32017, .T. ) ;
#93478=EDGE_LOOP ( 'NONE', ( #64120, #120602, #2591, #26119 ) ) ;
#93479=ORIENTED_EDGE ( 'NONE', *, *, #62068, .T. ) ;
#93480=AXIS2_PLACEMENT_3D ( 'NONE', #90181, #120315, #41128 ) ;
#93481=FACE_OUTER_BOUND ( 'NONE', #109353, .T. ) ;
#93482=CARTESIAN_POINT ( 'NONE',  ( -13.74999999999998934, 2.500000000000000000, 2.857883832488652853 ) ) ;
#93483=EDGE_CURVE ( 'NONE', #39312, #13198, #38370, .T. ) ;
#93484=CONICAL_SURFACE ( 'NONE', #3393, 0.09999999999999982514, 0.003490658503988666988 ) ;
#93485=ORIENTED_EDGE ( 'NONE', *, *, #53901, .F. ) ;
#93486=CYLINDRICAL_SURFACE ( 'NONE', #61123, 1.000000000000000888 ) ;
#93487=CIRCLE ( 'NONE', #68429, 0.09999999999999982514 ) ;
#93488=DIRECTION ( 'NONE',  ( -0.000000000000000000, -1.000000000000000000, -0.000000000000000000 ) ) ;
#93489=DIRECTION ( 'NONE',  ( 0.000000000000000000, 0.000000000000000000, -1.000000000000000000 ) ) ;
#93490=ORIENTED_EDGE ( 'NONE', *, *, #126407, .T. ) ;
#93491=DIRECTION ( 'NONE',  ( 0.000000000000000000, 0.000000000000000000, -1.000000000000000000 ) ) ;
#93492=DIRECTION ( 'NONE',  ( -0.000000000000000000, -1.000000000000000000, -0.000000000000000000 ) ) ;
#93493=EDGE_LOOP ( 'NONE', ( #50936, #36850, #65574, #111795 ) ) ;
#93494=VERTEX_POINT ( 'NONE', #129582 ) ;
#93495=ORIENTED_EDGE ( 'NONE', *, *, #89334, .T. ) ;
#93496=EDGE_LOOP ( 'NONE', ( #104172, #59046, #62437, #126124 ) ) ;
#93497=CARTESIAN_POINT ( 'NONE',  ( -6.850000000000017408, 12.50000000000000000, -6.841600689897077814 ) ) ;
#93498=AXIS2_PLACEMENT_3D ( 'NONE', #94196, #7084, #85661 ) ;
#93499=DIRECTION ( 'NONE',  ( -0.000000000000000000, 1.000000000000000000, -0.000000000000000000 ) ) ;
#93500=DIRECTION ( 'NONE',  ( -0.000000000000000000, 1.000000000000000000, -0.000000000000000000 ) ) ;
#93501=CARTESIAN_POINT ( 'NONE',  ( 11.24999999999990585, 2.500000000000000000, 2.957883832488649389 ) ) ;
#93502=VERTEX_POINT ( 'NONE', #21533 ) ;
#93503=DIRECTION ( 'NONE',  ( 0.000000000000000000, -0.000000000000000000, 1.000000000000000000 ) ) ;
#93504=ORIENTED_EDGE ( 'NONE', *, *, #33389, .T. ) ;
#93505=DIRECTION ( 'NONE',  ( -4.274815082592931898E-19, -0.9999939076577903929, -0.003490651415223739937 ) ) ;
#93506=DIRECTION ( 'NONE',  ( 0.000000000000000000, 1.000000000000000000, 0.000000000000000000 ) ) ;
#93507=DIRECTION ( 'NONE',  ( 0.000000000000000000, -0.9999939076577903929, 0.003490651415223739937 ) ) ;
#93508=DIRECTION ( 'NONE',  ( -0.000000000000000000, 1.000000000000000000, -0.000000000000000000 ) ) ;
#93509=VERTEX_POINT ( 'NONE', #32672 ) ;
#93510=AXIS2_PLACEMENT_3D ( 'NONE', #54148, #63966, #113053 ) ;
#93511=EDGE_CURVE ( 'NONE', #38170, #29262, #100722, .T. ) ;
#93512=CIRCLE ( 'NONE', #89400, 0.06509327318403745899 ) ;
#93513=ORIENTED_EDGE ( 'NONE', *, *, #19383, .T. ) ;
#93514=EDGE_LOOP ( 'NONE', ( #98074, #84888, #96288, #54445 ) ) ;
#93515=FACE_OUTER_BOUND ( 'NONE', #57725, .T. ) ;
#93516=DIRECTION ( 'NONE',  ( 0.000000000000000000, 0.000000000000000000, 1.000000000000000000 ) ) ;
#93517=CARTESIAN_POINT ( 'NONE',  ( -10.00000000000000355, 2.500000000000000000, 3.637306695894644726 ) ) ;
#93518=FACE_BOUND ( 'NONE', #7765, .T. ) ;
#93519=CARTESIAN_POINT ( 'NONE',  ( 5.399999999999931966, 2.500000000000000000, 4.330127018922196314 ) ) ;
#93520=DIRECTION ( 'NONE',  ( -4.274815082592931898E-19, -0.9999939076577903929, -0.003490651415223739937 ) ) ;
#93521=AXIS2_PLACEMENT_3D ( 'NONE', #29416, #10406, #120373 ) ;
#93522=FACE_OUTER_BOUND ( 'NONE', #13418, .T. ) ;
#93523=EDGE_CURVE ( 'NONE', #36055, #45761, #10419, .T. ) ;
#93524=CARTESIAN_POINT ( 'NONE',  ( 12.09999999999990550, 2.500000000000000000, -5.022947341949754119 ) ) ;
#93525=DIRECTION ( 'NONE',  ( 0.000000000000000000, 0.000000000000000000, 1.000000000000000000 ) ) ;
#93526=FACE_OUTER_BOUND ( 'NONE', #125729, .T. ) ;
#93527=ORIENTED_EDGE ( 'NONE', *, *, #103340, .T. ) ;
#93528=CONICAL_SURFACE ( 'NONE', #68477, 0.1000000000000000472, 0.003490658503988666988 ) ;
#93529=CIRCLE ( 'NONE', #32918, 0.06509327318403745899 ) ;
#93530=CONICAL_SURFACE ( 'NONE', #51770, 0.1000000000000002554, 0.003490658503988666988 ) ;
#93531=DIRECTION ( 'NONE',  ( -0.000000000000000000, -1.000000000000000000, -0.000000000000000000 ) ) ;
#93532=EDGE_LOOP ( 'NONE', ( #7711, #74492 ) ) ;
#93533=VERTEX_POINT ( 'NONE', #11048 ) ;
#93534=ORIENTED_EDGE ( 'NONE', *, *, #113353, .F. ) ;
#93535=ORIENTED_EDGE ( 'NONE', *, *, #68146, .T. ) ;
#93536=DIRECTION ( 'NONE',  ( 0.000000000000000000, 1.000000000000000000, 0.000000000000000000 ) ) ;
#93537=FACE_BOUND ( 'NONE', #123300, .T. ) ;
#93538=DIRECTION ( 'NONE',  ( 0.000000000000000000, 0.000000000000000000, 1.000000000000000000 ) ) ;
#93539=CONICAL_SURFACE ( 'NONE', #30863, 0.1000000000000002554, 0.003490658503988666988 ) ;
#93540=CIRCLE ( 'NONE', #104008, 0.09999999999999999167 ) ;
#93541=VERTEX_POINT ( 'NONE', #90250 ) ;
#93542=CARTESIAN_POINT ( 'NONE',  ( 59.88499455100932067, 2.860410828906190250, 5.641292085229139275 ) ) ;
#93543=DIRECTION ( 'NONE',  ( 0.000000000000000000, -0.9999939076577903929, 0.003490651415223739937 ) ) ;
#93544=AXIS2_PLACEMENT_3D ( 'NONE', #90836, #24522, #84073 ) ;
#93545=EDGE_LOOP ( 'NONE', ( #102657, #81981, #105171, #129351 ) ) ;
#93546=DIRECTION ( 'NONE',  ( 1.000000000000000000, 0.000000000000000000, 0.000000000000000000 ) ) ;
#93547=VECTOR ( 'NONE', #38471, 1000.000000000000000 ) ;
#93548=CARTESIAN_POINT ( 'NONE',  ( 1.649999999999951505, 2.500000000000000000, 1.472243186433545459 ) ) ;
#93549=ADVANCED_FACE ( 'NONE', ( #51013 ), #15339, .T. ) ;
#93550=CIRCLE ( 'NONE', #74778, 0.09999999999999982514 ) ;
#93551=ORIENTED_EDGE ( 'NONE', *, *, #35989, .T. ) ;
#93552=CARTESIAN_POINT ( 'NONE',  ( -0.4500000000000397571, 12.50000000000000000, -6.430097255199264339 ) ) ;
#93553=CARTESIAN_POINT ( 'NONE',  ( -13.09999999999999076, 12.50000000000000000, 3.983716857408420964 ) ) ;
#93554=AXIS2_PLACEMENT_3D ( 'NONE', #72323, #84048, #104346 ) ;
#93555=CIRCLE ( 'NONE', #95715, 0.06509327318403745899 ) ;
#93556=ADVANCED_FACE ( 'NONE', ( #11706 ), #84313, .T. ) ;
#93557=ORIENTED_EDGE ( 'NONE', *, *, #23697, .T. ) ;
#93558=CONICAL_SURFACE ( 'NONE', #72638, 0.1000000000000000472, 0.003490658503988666988 ) ;
#93559=AXIS2_PLACEMENT_3D ( 'NONE', #64187, #43926, #34754 ) ;
#93560=LINE ( 'NONE', #46374, #55127 ) ;
#93561=B_SPLINE_CURVE_WITH_KNOTS ( 'NONE', 3,
 ( #96719, #7043, #58749, #47001, #128135, #117634, #67912, #86905 ),
 .UNSPECIFIED., .F., .F.,
 ( 4, 2, 2, 4 ),
 ( -0.0001155885020466859676, 0.03307027595371006545, 0.04966320818158844602, 0.06625614040946682659 ),
 .UNSPECIFIED. ) ;
#93562=CARTESIAN_POINT ( 'NONE',  ( 4.599999999999937472, 2.500000000000000000, 0.5928203230275495006 ) ) ;
#93563=CARTESIAN_POINT ( 'NONE',  ( -8.750000000000007105, 2.500000000000000000, 7.188010851410848723 ) ) ;
#93564=EDGE_LOOP ( 'NONE', ( #67646, #44165 ) ) ;
#93565=ADVANCED_FACE ( 'NONE', ( #20890 ), #103096, .T. ) ;
#93566=ORIENTED_EDGE ( 'NONE', *, *, #49763, .T. ) ;
#93567=EDGE_CURVE ( 'NONE', #12736, #118052, #72577, .T. ) ;
#93568=CARTESIAN_POINT ( 'NONE',  ( -6.050000000000018474, 2.500000000000000000, 6.941600689897073018 ) ) ;
#93569=EDGE_LOOP ( 'NONE', ( #55930, #111397, #12174, #432 ) ) ;
#93570=CARTESIAN_POINT ( 'NONE',  ( 2.299999999999948752, 2.500000000000000000, 0.2464101615137735679 ) ) ;
#93571=DIRECTION ( 'NONE',  ( -4.274815082592931898E-19, -0.9999939076577903929, -0.003490651415223739937 ) ) ;
#93572=AXIS2_PLACEMENT_3D ( 'NONE', #40825, #81388, #82676 ) ;
#93573=AXIS2_PLACEMENT_3D ( 'NONE', #16526, #76116, #77405 ) ;
#93574=VERTEX_POINT ( 'NONE', #71938 ) ;
#93575=EDGE_CURVE ( 'NONE', #96273, #1760, #55071, .T. ) ;
#93576=DIRECTION ( 'NONE',  ( -0.000000000000000000, -1.000000000000000000, -0.000000000000000000 ) ) ;
#93577=DIRECTION ( 'NONE',  ( 0.000000000000000000, 0.000000000000000000, -1.000000000000000000 ) ) ;
#93578=DIRECTION ( 'NONE',  ( 0.000000000000000000, 0.000000000000000000, -1.000000000000000000 ) ) ;
#93579=DIRECTION ( 'NONE',  ( 0.000000000000000000, 1.000000000000000000, 0.000000000000000000 ) ) ;
#93580=EDGE_CURVE ( 'NONE', #27907, #9598, #112498, .T. ) ;
#93581=LINE ( 'NONE', #112583, #26519 ) ;
#93582=VERTEX_POINT ( 'NONE', #22199 ) ;
#93583=ORIENTED_EDGE ( 'NONE', *, *, #44168, .F. ) ;
#93584=CARTESIAN_POINT ( 'NONE',  ( -3.550000000000028688, 2.500000000000000000, 6.941600689897073018 ) ) ;
#93585=CARTESIAN_POINT ( 'NONE',  ( -14.34999999999998543, 12.50000000000000000, 1.883746621131362931 ) ) ;
#93587=ORIENTED_EDGE ( 'NONE', *, *, #63597, .F. ) ;
#93588=EDGE_LOOP ( 'NONE', ( #94659, #68114, #124790, #97468 ) ) ;
#93590=DIRECTION ( 'NONE',  ( 0.000000000000000000, -0.9999939076577903929, 0.003490651415223739937 ) ) ;
#93591=DIRECTION ( 'NONE',  ( 0.000000000000000000, 1.000000000000000000, 0.000000000000000000 ) ) ;
#93592=DIRECTION ( 'NONE',  ( -0.000000000000000000, -1.000000000000000000, -0.000000000000000000 ) ) ;
#93593=DIRECTION ( 'NONE',  ( 0.000000000000000000, 1.000000000000000000, 0.000000000000000000 ) ) ;
#93594=FACE_OUTER_BOUND ( 'NONE', #30795, .T. ) ;
#93595=FACE_OUTER_BOUND ( 'NONE', #119052, .T. ) ;
#93596=DIRECTION ( 'NONE',  ( -0.000000000000000000, 1.000000000000000000, -0.000000000000000000 ) ) ;
#93597=CARTESIAN_POINT ( 'NONE',  ( 2.099999999999950351, 12.50000000000000000, -2.276824562219559311E-15 ) ) ;
#93598=CARTESIAN_POINT ( 'NONE',  ( -2.950000000000029932, 2.500000000000000000, -2.265063509461101798 ) ) ;
#93599=AXIS2_PLACEMENT_3D ( 'NONE', #8096, #7446, #87931 ) ;
#93600=ORIENTED_EDGE ( 'NONE', *, *, #9797, .F. ) ;
#93601=EDGE_CURVE ( 'NONE', #11848, #128991, #121979, .T. ) ;
#93602=CIRCLE ( 'NONE', #26704, 0.06509327318403745899 ) ;
#93603=CARTESIAN_POINT ( 'NONE',  ( -4.600000000000025402, 12.50000000000000000, 4.330127018922196314 ) ) ;
#93604=EDGE_LOOP ( 'NONE', ( #28066, #33688, #57192, #83673 ) ) ;
#93605=EDGE_LOOP ( 'NONE', ( #95796, #76058 ) ) ;
#93606=CARTESIAN_POINT ( 'NONE',  ( 8.149999999999923972, 2.500000000000000000, -6.741600689897077281 ) ) ;
#93607=DIRECTION ( 'NONE',  ( 0.000000000000000000, 0.000000000000000000, 1.000000000000000000 ) ) ;
#93608=FACE_OUTER_BOUND ( 'NONE', #27873, .T. ) ;
#93609=CONICAL_SURFACE ( 'NONE', #32987, 0.1000000000000002554, 0.003490658503988666988 ) ;
#93610=EDGE_CURVE ( 'NONE', #29262, #50768, #126174, .T. ) ;
#93611=DIRECTION ( 'NONE',  ( 0.000000000000000000, 1.000000000000000000, 0.000000000000000000 ) ) ;
#93612=AXIS2_PLACEMENT_3D ( 'NONE', #1983, #41933, #100821 ) ;
#93613=AXIS2_PLACEMENT_3D ( 'NONE', #86645, #109515, #68936 ) ;
#93614=CARTESIAN_POINT ( 'NONE',  ( 8.749999999999918288, 12.50000000000000000, -1.472243186433550122 ) ) ;
#93616=DIRECTION ( 'NONE',  ( 0.000000000000000000, 0.000000000000000000, 1.000000000000000000 ) ) ;
#93617=VERTEX_POINT ( 'NONE', #121021 ) ;
#93618=CARTESIAN_POINT ( 'NONE',  ( -2.100000000000034728, 12.50000000000000000, 4.265033745738159077 ) ) ;
#93619=EDGE_CURVE ( 'NONE', #27240, #48072, #19569, .T. ) ;
#93620=EDGE_CURVE ( 'NONE', #54758, #51555, #128251, .T. ) ;
#93621=ADVANCED_FACE ( 'NONE', ( #43770 ), #34149, .T. ) ;
#93622=CARTESIAN_POINT ( 'NONE',  ( -7.900000000000014566, 12.50000000000000000, -5.022947341949754119 ) ) ;
#93623=ORIENTED_EDGE ( 'NONE', *, *, #88840, .T. ) ;
#93624=CIRCLE ( 'NONE', #49727, 0.1000000000000000472 ) ;
#93625=VERTEX_POINT ( 'NONE', #94133 ) ;
#93626=ADVANCED_FACE ( 'NONE', ( #65960 ), #44389, .T. ) ;
#93627=ORIENTED_EDGE ( 'NONE', *, *, #28334, .F. ) ;
#93628=CIRCLE ( 'NONE', #110348, 0.09999999999999982514 ) ;
#93629=VERTEX_POINT ( 'NONE', #14274 ) ;
#93630=CARTESIAN_POINT ( 'NONE',  ( 4.599999999999940137, 2.500000000000000000, -4.430127018922202176 ) ) ;
#93631=DIRECTION ( 'NONE',  ( 0.000000000000000000, 1.000000000000000000, 0.000000000000000000 ) ) ;
#93632=ADVANCED_FACE ( 'NONE', ( #83046 ), #9098, .T. ) ;
#93633=AXIS2_PLACEMENT_3D ( 'NONE', #112680, #46340, #126200 ) ;
#93634=EDGE_CURVE ( 'NONE', #109159, #31303, #54220, .T. ) ;
#93635=DIRECTION ( 'NONE',  ( 0.000000000000000000, 1.000000000000000000, 0.000000000000000000 ) ) ;
#93636=CARTESIAN_POINT ( 'NONE',  ( -4.400000000000025224, 2.500000000000000000, 0.2464101615137735679 ) ) ;
#93637=CIRCLE ( 'NONE', #95777, 0.06509327318403745899 ) ;
#93638=DIRECTION ( 'NONE',  ( -0.000000000000000000, -1.000000000000000000, -0.000000000000000000 ) ) ;
#93639=EDGE_LOOP ( 'NONE', ( #112673, #77641 ) ) ;
#93640=CARTESIAN_POINT ( 'NONE',  ( 2.099999999999950351, 12.50000000000000000, -0.6928203230275541413 ) ) ;
#93641=DIRECTION ( 'NONE',  ( -0.000000000000000000, 1.000000000000000000, -0.000000000000000000 ) ) ;
#93642=CARTESIAN_POINT ( 'NONE',  ( -9.350000000000006750, 12.50000000000000000, 2.446380397790835826 ) ) ;
#93643=VECTOR ( 'NONE', #73453, 1000.000000000000000 ) ;
#93644=CONICAL_SURFACE ( 'NONE', #70653, 0.09999999999999982514, 0.003490658503988666988 ) ;
#93645=FACE_OUTER_BOUND ( 'NONE', #111324, .T. ) ;
#93646=VERTEX_POINT ( 'NONE', #115045 ) ;
#93647=VECTOR ( 'NONE', #46018, 1000.000000000000000 ) ;
#93648=EDGE_LOOP ( 'NONE', ( #100280, #112698, #108576, #70385 ) ) ;
#93649=ORIENTED_EDGE ( 'NONE', *, *, #68329, .F. ) ;
#93650=DIRECTION ( 'NONE',  ( 0.000000000000000000, 1.000000000000000000, 0.000000000000000000 ) ) ;
#93651=AXIS2_PLACEMENT_3D ( 'NONE', #55880, #37551, #56523 ) ;
#93652=VECTOR ( 'NONE', #39506, 1000.000000000000000 ) ;
#93653=CARTESIAN_POINT ( 'NONE',  ( 2.099999999999950351, 12.50000000000000000, -0.6277270498435166823 ) ) ;
#93654=DIRECTION ( 'NONE',  ( 0.000000000000000000, 1.000000000000000000, 0.000000000000000000 ) ) ;
#93655=AXIS2_PLACEMENT_3D ( 'NONE', #6373, #86896, #125532 ) ;
#93656=VERTEX_POINT ( 'NONE', #55507 ) ;
#93657=DIRECTION ( 'NONE',  ( -0.000000000000000000, 1.000000000000000000, -0.000000000000000000 ) ) ;
#93658=DIRECTION ( 'NONE',  ( -0.000000000000000000, 1.000000000000000000, -0.000000000000000000 ) ) ;
#93659=AXIS2_PLACEMENT_3D ( 'NONE', #117018, #98045, #96110 ) ;
#93660=PLANE ( 'NONE',  #10642 ) ;
#93661=DIRECTION ( 'NONE',  ( 0.000000000000000000, -0.9999939076577903929, 0.003490651415223739937 ) ) ;
#93662=CONICAL_SURFACE ( 'NONE', #104128, 0.1000000000000002554, 0.003490658503988666988 ) ;
#93663=CYLINDRICAL_SURFACE ( 'NONE', #3935, 2.000000000000000000 ) ;
#93664=EDGE_CURVE ( 'NONE', #76363, #115754, #43134, .T. ) ;
#93665=VERTEX_POINT ( 'NONE', #124250 ) ;
#93666=ORIENTED_EDGE ( 'NONE', *, *, #21332, .F. ) ;
#93668=DIRECTION ( 'NONE',  ( -0.000000000000000000, -1.000000000000000000, -0.000000000000000000 ) ) ;
#93669=DIRECTION ( 'NONE',  ( 0.000000000000000000, 0.000000000000000000, -1.000000000000000000 ) ) ;
#93670=CARTESIAN_POINT ( 'NONE',  ( 9.349999999999919709, 2.500000000000000000, 1.718653347947321386 ) ) ;
#93671=DIRECTION ( 'NONE',  ( 0.000000000000000000, 0.000000000000000000, 1.000000000000000000 ) ) ;
#93672=EDGE_CURVE ( 'NONE', #98954, #56105, #63393, .T. ) ;
#93673=ORIENTED_EDGE ( 'NONE', *, *, #79401, .F. ) ;
#93674=ORIENTED_EDGE ( 'NONE', *, *, #32846, .T. ) ;
#93675=DIRECTION ( 'NONE',  ( 0.000000000000000000, 0.000000000000000000, 1.000000000000000000 ) ) ;
#93676=DIRECTION ( 'NONE',  ( 0.000000000000000000, -0.9999939076577903929, 0.003490651415223739937 ) ) ;
#93677=CARTESIAN_POINT ( 'NONE',  ( 17.46224641144930345, -2.500000000000000000, -5.244174873161000505 ) ) ;
#93679=EDGE_LOOP ( 'NONE', ( #10678, #115103 ) ) ;
#93680=CARTESIAN_POINT ( 'NONE',  ( 8.149999999999920419, 2.500000000000000000, 6.741600689897071952 ) ) ;
#93681=CARTESIAN_POINT ( 'NONE',  ( -6.850000000000017408, 2.500000000000000000, -1.818653347947325916 ) ) ;
#93682=AXIS2_PLACEMENT_3D ( 'NONE', #673, #111928, #40636 ) ;
#93683=CIRCLE ( 'NONE', #18465, 0.1000000000000000472 ) ;
#93684=EDGE_LOOP ( 'NONE', ( #31261, #100551 ) ) ;
#93685=AXIS2_PLACEMENT_3D ( 'NONE', #93403, #80373, #21431 ) ;
#93686=CARTESIAN_POINT ( 'NONE',  ( -5.450000000000023270, 2.500000000000000000, -6.495190528383302464 ) ) ;
#93687=VERTEX_POINT ( 'NONE', #84312 ) ;
#93688=CARTESIAN_POINT ( 'NONE',  ( 8.099999999999923261, 12.50000000000000000, 4.676537180435972552 ) ) ;
#93689=AXIS2_PLACEMENT_3D ( 'NONE', #30999, #72831, #83304 ) ;
#93690=CONICAL_SURFACE ( 'NONE', #10166, 0.09999999999999999167, 0.003490658503988666988 ) ;
#93691=ORIENTED_EDGE ( 'NONE', *, *, #24708, .F. ) ;
#93692=FACE_OUTER_BOUND ( 'NONE', #34820, .T. ) ;
#93693=PLANE ( 'NONE',  #92014 ) ;
#93695=ORIENTED_EDGE ( 'NONE', *, *, #103081, .F. ) ;
#93697=CARTESIAN_POINT ( 'NONE',  ( -10.65000000000000391, 12.50000000000000000, -6.213873640053560798 ) ) ;
#93698=CONICAL_SURFACE ( 'NONE', #53997, 0.1000000000000002554, 0.003490658503988666988 ) ;
#93699=DIRECTION ( 'NONE',  ( -0.000000000000000000, 1.000000000000000000, -0.000000000000000000 ) ) ;
#93701=CONICAL_SURFACE ( 'NONE', #16314, 0.09999999999999982514, 0.003490658503988666988 ) ;
#93702=DIRECTION ( 'NONE',  ( 0.000000000000000000, 1.000000000000000000, 0.000000000000000000 ) ) ;
#93703=DIRECTION ( 'NONE',  ( 0.000000000000000000, 0.000000000000000000, 1.000000000000000000 ) ) ;
#93704=DIRECTION ( 'NONE',  ( 0.000000000000000000, 1.000000000000000000, 0.000000000000000000 ) ) ;
#93705=FACE_OUTER_BOUND ( 'NONE', #44957, .T. ) ;
#93706=AXIS2_PLACEMENT_3D ( 'NONE', #117037, #37230, #8385 ) ;
#93707=EDGE_CURVE ( 'NONE', #97182, #98382, #114413, .T. ) ;
#93708=EDGE_LOOP ( 'NONE', ( #95371, #65754, #95138, #34160 ) ) ;
#93709=EDGE_LOOP ( 'NONE', ( #73171, #14362 ) ) ;
#93710=DIRECTION ( 'NONE',  ( 0.000000000000000000, 0.000000000000000000, 1.000000000000000000 ) ) ;
#93711=ORIENTED_EDGE ( 'NONE', *, *, #109698, .F. ) ;
#93712=FACE_OUTER_BOUND ( 'NONE', #3873, .T. ) ;
#93713=DIRECTION ( 'NONE',  ( -0.000000000000000000, -1.000000000000000000, -0.000000000000000000 ) ) ;
#93714=CIRCLE ( 'NONE', #95770, 0.1000000000000002554 ) ;
#93715=CARTESIAN_POINT ( 'NONE',  ( 7.499999999999925393, 2.500000000000000000, -0.6928203230275541413 ) ) ;
#93716=EDGE_LOOP ( 'NONE', ( #46999, #112789, #123768, #25315 ) ) ;
#93717=ORIENTED_EDGE ( 'NONE', *, *, #17806, .T. ) ;
#93718=ADVANCED_FACE ( 'NONE', ( #54840 ), #35866, .T. ) ;
#93719=FACE_BOUND ( 'NONE', #23391, .T. ) ;
#93720=VERTEX_POINT ( 'NONE', #24761 ) ;
#93721=EDGE_CURVE ( 'NONE', #89399, #110447, #92733, .T. ) ;
#93722=DIRECTION ( 'NONE',  ( 0.000000000000000000, -0.000000000000000000, 1.000000000000000000 ) ) ;
#93723=CARTESIAN_POINT ( 'NONE',  ( 4.549999999999939426, 12.50000000000000000, -6.495190528383302464 ) ) ;
#93724=ORIENTED_EDGE ( 'NONE', *, *, #53680, .F. ) ;
#93725=CARTESIAN_POINT ( 'NONE',  ( 1.249999999999950262, 2.500000000000000000, 7.088010851410848190 ) ) ;
#93726=CIRCLE ( 'NONE', #95775, 0.09999999999999982514 ) ;
#93727=DIRECTION ( 'NONE',  ( 0.000000000000000000, 0.000000000000000000, -1.000000000000000000 ) ) ;
#93728=CARTESIAN_POINT ( 'NONE',  ( -2.100000000000034284, 12.50000000000000000, 0.06509327318403504425 ) ) ;
#93729=CARTESIAN_POINT ( 'NONE',  ( -4.150000000000027889, 2.500000000000000000, -7.188010851410854052 ) ) ;
#93730=EDGE_CURVE ( 'NONE', #112512, #120557, #107298, .T. ) ;
#93731=DIRECTION ( 'NONE',  ( -4.274815082592931898E-19, -0.9999939076577903929, -0.003490651415223739937 ) ) ;
#93732=ADVANCED_FACE ( 'NONE', ( #53580 ), #98986, .T. ) ;
#93733=CARTESIAN_POINT ( 'NONE',  ( -9.150000000000005684, 12.50000000000000000, 6.495190528383297135 ) ) ;
#93735=CARTESIAN_POINT ( 'NONE',  ( 11.24999999999991118, 2.500000000000000000, 5.902370205355745192 ) ) ;
#93736=ADVANCED_FACE ( 'NONE', ( #5099 ), #36313, .T. ) ;
#93737=CIRCLE ( 'NONE', #37312, 0.1000000000000000056 ) ;
#93738=DIRECTION ( 'NONE',  ( 0.000000000000000000, 0.000000000000000000, 1.000000000000000000 ) ) ;
#93740=CIRCLE ( 'NONE', #118771, 0.06509327318403745899 ) ;
#93741=ORIENTED_EDGE ( 'NONE', *, *, #97547, .F. ) ;
#93742=ORIENTED_EDGE ( 'NONE', *, *, #35976, .T. ) ;
#93743=DIRECTION ( 'NONE',  ( 0.000000000000000000, 0.000000000000000000, -1.000000000000000000 ) ) ;
#93744=EDGE_LOOP ( 'NONE', ( #5900, #22215 ) ) ;
#93745=ORIENTED_EDGE ( 'NONE', *, *, #124203, .T. ) ;
#93746=ORIENTED_EDGE ( 'NONE', *, *, #68774, .T. ) ;
#93747=ORIENTED_EDGE ( 'NONE', *, *, #88459, .F. ) ;
#93748=AXIS2_PLACEMENT_3D ( 'NONE', #112726, #23051, #14493 ) ;
#93749=DIRECTION ( 'NONE',  ( 0.000000000000000000, -0.000000000000000000, 1.000000000000000000 ) ) ;
#93750=FACE_OUTER_BOUND ( 'NONE', #5730, .T. ) ;
#93752=CARTESIAN_POINT ( 'NONE',  ( 5.399999999999932854, 2.500000000000000000, 3.637306695894644726 ) ) ;
#93753=DIRECTION ( 'NONE',  ( 0.000000000000000000, -0.9999939076577903929, 0.003490651415223739937 ) ) ;
#93754=LINE ( 'NONE', #83918, #60089 ) ;
#93755=CIRCLE ( 'NONE', #58167, 0.1000000000000000472 ) ;
#93756=EDGE_LOOP ( 'NONE', ( #93587, #56381, #113587, #52752 ) ) ;
#93757=DIRECTION ( 'NONE',  ( 0.000000000000000000, 0.000000000000000000, 1.000000000000000000 ) ) ;
#93758=VERTEX_POINT ( 'NONE', #64035 ) ;
#93759=AXIS2_PLACEMENT_3D ( 'NONE', #84916, #94729, #65259 ) ;
#93760=CIRCLE ( 'NONE', #47789, 0.06509327318403745899 ) ;
#93761=ORIENTED_EDGE ( 'NONE', *, *, #80209, .T. ) ;
#93762=ORIENTED_EDGE ( 'NONE', *, *, #13503, .T. ) ;
#93763=CARTESIAN_POINT ( 'NONE',  ( -14.99999999999998224, 2.500000000000000000, -0.6928203230275519209 ) ) ;
#93764=( BOUNDED_SURFACE ( )  B_SPLINE_SURFACE ( 3, 2, ( 
 ( #32681, #62123, #45066 ),
 ( #84965, #124897, #22207 ),
 ( #112508, #12985, #74508 ),
 ( #72585, #52938, #43143 ),
 ( #83053, #33315, #73224 ),
 ( #43780, #24123, #73859 ),
 ( #33943, #113138, #113795 ),
 ( #64044, #103974, #4442 ),
 ( #94144, #17500, #97366 ),
 ( #26056, #116986, #106536 ),
 ( #37803, #37175, #35875 ),
 ( #55519, #86239, #85609 ),
 ( #77710, #8332, #48266 ),
 ( #88162, #95441, #127478 ),
 ( #98003, #115707, #46992 ),
 ( #67222, #46328, #16205 ) ),
 .UNSPECIFIED., .F., .F., .F. ) 
 B_SPLINE_SURFACE_WITH_KNOTS ( ( 4, 2, 2, 2, 2, 2, 2, 4 ),
 ( 3, 3 ),
 ( 0.000000000000000000, 0.003502803217043997872, 0.007005606434087995743, 0.008757008042609995546, 0.01050840965113199361, 0.01225981125965399168, 0.01313551206391499158, 0.01401121286817599149 ),
 ( 0.000000000000000000, 1.000000000000000000 ),
 .UNSPECIFIED. ) 
 GEOMETRIC_REPRESENTATION_ITEM ( )  RATIONAL_B_SPLINE_SURFACE ( (
 ( 1.000000000000000000, 0.7071067811865476838, 1.000000000000000000),
 ( 1.000000000000000000, 0.7071067811865476838, 1.000000000000000000),
 ( 1.000000000000000000, 0.7071067811865474617, 1.000000000000000000),
 ( 1.000000000000000000, 0.7071067811865474617, 1.000000000000000000),
 ( 1.000000000000000000, 0.7071067811865477948, 1.000000000000000000),
 ( 1.000000000000000000, 0.7071067811865477948, 1.000000000000000000),
 ( 1.000000000000000000, 0.7071067811865473507, 1.000000000000000000),
 ( 1.000000000000000000, 0.7071067811865473507, 1.000000000000000000),
 ( 1.000000000000000000, 0.7071067811865472397, 1.000000000000000000),
 ( 1.000000000000000000, 0.7071067811865472397, 1.000000000000000000),
 ( 1.000000000000000000, 0.7071067811865473507, 1.000000000000000000),
 ( 1.000000000000000000, 0.7071067811865473507, 1.000000000000000000),
 ( 1.000000000000000000, 0.7071067811865472397, 1.000000000000000000),
 ( 1.000000000000000000, 0.7071067811865472397, 1.000000000000000000),
 ( 1.000000000000000000, 0.7071067811865479058, 1.000000000000000000),
 ( 1.000000000000000000, 0.7071067811865479058, 1.000000000000000000) ) ) 
 REPRESENTATION_ITEM ( '' )  SURFACE ( )  );
#93765=ORIENTED_EDGE ( 'NONE', *, *, #75285, .T. ) ;
#93766=ORIENTED_EDGE ( 'NONE', *, *, #51786, .T. ) ;
#93767=EDGE_LOOP ( 'NONE', ( #41173, #120231, #126673, #8803 ) ) ;
#93768=PLANE ( 'NONE',  #88430 ) ;
#93769=CARTESIAN_POINT ( 'NONE',  ( -6.450000000000014388, 2.500000000000000000, 1.818653347947321475 ) ) ;
#93770=DIRECTION ( 'NONE',  ( -4.274815082592931898E-19, -0.9999939076577903929, -0.003490651415223739937 ) ) ;
#93771=DIRECTION ( 'NONE',  ( 0.000000000000000000, 1.000000000000000000, 0.000000000000000000 ) ) ;
#93773=EDGE_CURVE ( 'NONE', #4955, #103364, #29949, .T. ) ;
#93774=DIRECTION ( 'NONE',  ( 0.000000000000000000, -0.9999939076577903929, 0.003490651415223739937 ) ) ;
#93775=VECTOR ( 'NONE', #11098, 1000.000000000000000 ) ;
#93776=EDGE_CURVE ( 'NONE', #127507, #116228, #45691, .T. ) ;
#93777=EDGE_CURVE ( 'NONE', #55129, #89331, #101043, .T. ) ;
#93778=DIRECTION ( 'NONE',  ( 0.000000000000000000, -0.9999939076577903929, 0.003490651415223739937 ) ) ;
#93779=ORIENTED_EDGE ( 'NONE', *, *, #91944, .F. ) ;
#93780=CONICAL_SURFACE ( 'NONE', #5916, 0.09999999999999982514, 0.003490658503988666988 ) ;
#93781=CARTESIAN_POINT ( 'NONE',  ( -12.89999999999999325, 12.50000000000000000, -3.637306695894647390 ) ) ;
#93782=CIRCLE ( 'NONE', #62489, 0.09999999999999999167 ) ;
#93783=EDGE_LOOP ( 'NONE', ( #38339, #38895, #94462, #202 ) ) ;
#93784=DIRECTION ( 'NONE',  ( 0.000000000000000000, 0.000000000000000000, 1.000000000000000000 ) ) ;
#93785=VECTOR ( 'NONE', #81048, 1000.000000000000000 ) ;
#93786=ADVANCED_FACE ( 'NONE', ( #6364 ), #40426, .T. ) ;
#93787=EDGE_CURVE ( 'NONE', #34238, #8778, #18786, .T. ) ;
#93788=ORIENTED_EDGE ( 'NONE', *, *, #39800, .T. ) ;
#93789=ORIENTED_EDGE ( 'NONE', *, *, #53088, .T. ) ;
#93790=AXIS2_PLACEMENT_3D ( 'NONE', #72345, #110317, #82151 ) ;
#93791=CARTESIAN_POINT ( 'NONE',  ( -1.700000000000034817, 2.500000000000000000, -4.330127018922201643 ) ) ;
#93792=DIRECTION ( 'NONE',  ( -4.274815082592931898E-19, -0.9999939076577903929, -0.003490651415223739937 ) ) ;
#93793=AXIS2_PLACEMENT_3D ( 'NONE', #83150, #123065, #104690 ) ;
#93794=ADVANCED_FACE ( 'NONE', ( #7671 ), #21630, .T. ) ;
#93795=AXIS2_PLACEMENT_3D ( 'NONE', #106476, #56077, #14842 ) ;
#93796=ADVANCED_FACE ( 'NONE', ( #17490 ), #124022, .T. ) ;
#93797=PLANE ( 'NONE',  #92495 ) ;
#93798=ORIENTED_EDGE ( 'NONE', *, *, #100673, .F. ) ;
#93799=ORIENTED_EDGE ( 'NONE', *, *, #127724, .T. ) ;
#93800=DIRECTION ( 'NONE',  ( -0.000000000000000000, 1.000000000000000000, -0.000000000000000000 ) ) ;
#93801=DIRECTION ( 'NONE',  ( 0.000000000000000000, -0.9999939076577903929, 0.003490651415223739937 ) ) ;
#93802=DIRECTION ( 'NONE',  ( 0.000000000000000000, 1.000000000000000000, 0.000000000000000000 ) ) ;
#93803=DIRECTION ( 'NONE',  ( 0.000000000000000000, -0.000000000000000000, 1.000000000000000000 ) ) ;
#93804=EDGE_CURVE ( 'NONE', #99888, #43212, #57122, .T. ) ;
#93805=AXIS2_PLACEMENT_3D ( 'NONE', #99165, #67760, #107692 ) ;
#93806=DIRECTION ( 'NONE',  ( 0.000000000000000000, -0.000000000000000000, 1.000000000000000000 ) ) ;
#93807=VECTOR ( 'NONE', #115840, 1000.000000000000000 ) ;
#93808=ORIENTED_EDGE ( 'NONE', *, *, #31272, .T. ) ;
#93809=ORIENTED_EDGE ( 'NONE', *, *, #46021, .T. ) ;
#93810=DIRECTION ( 'NONE',  ( 0.000000000000000000, 0.000000000000000000, -1.000000000000000000 ) ) ;
#93811=DIRECTION ( 'NONE',  ( 0.000000000000000000, 0.000000000000000000, 1.000000000000000000 ) ) ;
#93812=CONICAL_SURFACE ( 'NONE', #31134, 0.1000000000000002554, 0.003490658503988666988 ) ;
#93813=AXIS2_PLACEMENT_3D ( 'NONE', #72079, #110060, #11840 ) ;
#93815=FACE_OUTER_BOUND ( 'NONE', #11831, .T. ) ;
#93816=DIRECTION ( 'NONE',  ( 0.000000000000000000, -0.000000000000000000, 1.000000000000000000 ) ) ;
#93817=DIRECTION ( 'NONE',  ( 0.000000000000000000, -0.000000000000000000, 1.000000000000000000 ) ) ;
#93818=DIRECTION ( 'NONE',  ( 0.000000000000000000, 1.000000000000000000, 0.000000000000000000 ) ) ;
#93819=ORIENTED_EDGE ( 'NONE', *, *, #67748, .F. ) ;
#93820=DIRECTION ( 'NONE',  ( 0.000000000000000000, -0.000000000000000000, 1.000000000000000000 ) ) ;
#93821=DIRECTION ( 'NONE',  ( 0.000000000000000000, 0.000000000000000000, 1.000000000000000000 ) ) ;
#93822=DIRECTION ( 'NONE',  ( 0.000000000000000000, 0.000000000000000000, -1.000000000000000000 ) ) ;
#93823=CIRCLE ( 'NONE', #118943, 0.1000000000000002554 ) ;
#93824=ORIENTED_EDGE ( 'NONE', *, *, #109997, .T. ) ;
#93825=CIRCLE ( 'NONE', #16432, 0.06509327318403745899 ) ;
#93826=CARTESIAN_POINT ( 'NONE',  ( 11.89999999999990798, 12.50000000000000000, 4.741630453620009789 ) ) ;
#93827=AXIS2_PLACEMENT_3D ( 'NONE', #102817, #13142, #53096 ) ;
#93828=EDGE_CURVE ( 'NONE', #22216, #78336, #21720, .T. ) ;
#93829=ORIENTED_EDGE ( 'NONE', *, *, #1749, .F. ) ;
#93830=DIRECTION ( 'NONE',  ( 0.000000000000000000, 0.000000000000000000, -1.000000000000000000 ) ) ;
#93831=ORIENTED_EDGE ( 'NONE', *, *, #63280, .T. ) ;
#93832=CARTESIAN_POINT ( 'NONE',  ( 5.399999999999935518, 2.500000000000000000, -4.430127018922202176 ) ) ;
#93833=VECTOR ( 'NONE', #15965, 1000.000000000000000 ) ;
#93834=DIRECTION ( 'NONE',  ( -0.000000000000000000, -1.000000000000000000, -0.000000000000000000 ) ) ;
#93835=CARTESIAN_POINT ( 'NONE',  ( 13.14999999999990088, 2.500000000000000000, 2.511473670974873507 ) ) ;
#93836=VERTEX_POINT ( 'NONE', #47620 ) ;
#93837=CARTESIAN_POINT ( 'NONE',  ( -10.85000000000000142, 2.500000000000000000, -1.572243186433546214 ) ) ;
#93838=AXIS2_PLACEMENT_3D ( 'NONE', #90395, #70143, #736 ) ;
#93839=AXIS2_PLACEMENT_3D ( 'NONE', #129604, #120410, #71287 ) ;
#93840=DIRECTION ( 'NONE',  ( 0.000000000000000000, 1.000000000000000000, 0.000000000000000000 ) ) ;
#93841=CONICAL_SURFACE ( 'NONE', #125148, 0.1000000000000002554, 0.003490658503988666988 ) ;
#93842=VERTEX_POINT ( 'NONE', #108458 ) ;
#93843=DIRECTION ( 'NONE',  ( 0.000000000000000000, 0.000000000000000000, -1.000000000000000000 ) ) ;
#93844=CONICAL_SURFACE ( 'NONE', #100205, 0.1000000000000000472, 0.003490658503988666988 ) ;
#93845=CIRCLE ( 'NONE', #114761, 0.06509327318403745899 ) ;
#93846=ORIENTED_EDGE ( 'NONE', *, *, #48638, .T. ) ;
#93847=VERTEX_POINT ( 'NONE', #98626 ) ;
#93848=FACE_OUTER_BOUND ( 'NONE', #63214, .T. ) ;
#93849=CARTESIAN_POINT ( 'NONE',  ( -13.74999999999998934, 2.500000000000000000, 2.857883832488652853 ) ) ;
#93850=CARTESIAN_POINT ( 'NONE',  ( -3.550000000000027800, 2.500000000000000000, 6.148780366869520009 ) ) ;
#93851=VERTEX_POINT ( 'NONE', #28629 ) ;
#93852=CARTESIAN_POINT ( 'NONE',  ( 13.34999999999989662, 2.500000000000000000, -2.265063509461101798 ) ) ;
#93853=CARTESIAN_POINT ( 'NONE',  ( -0.8500000000000386136, 12.50000000000000000, 7.188010851410848723 ) ) ;
#93854=ORIENTED_EDGE ( 'NONE', *, *, #57893, .F. ) ;
#93855=DIRECTION ( 'NONE',  ( 0.000000000000000000, 0.000000000000000000, -1.000000000000000000 ) ) ;
#93856=DIRECTION ( 'NONE',  ( 0.000000000000000000, 0.000000000000000000, 1.000000000000000000 ) ) ;
#93857=DIRECTION ( 'NONE',  ( 0.000000000000000000, -0.9999939076577903929, 0.003490651415223739937 ) ) ;
#93858=DIRECTION ( 'NONE',  ( -0.000000000000000000, -1.000000000000000000, -0.000000000000000000 ) ) ;
#93859=VECTOR ( 'NONE', #114465, 1000.000000000000000 ) ;
#93860=FACE_OUTER_BOUND ( 'NONE', #931, .T. ) ;
#93861=DIRECTION ( 'NONE',  ( 0.000000000000000000, 0.000000000000000000, 1.000000000000000000 ) ) ;
#93862=DIRECTION ( 'NONE',  ( 0.000000000000000000, 0.000000000000000000, 1.000000000000000000 ) ) ;
#93863=AXIS2_PLACEMENT_3D ( 'NONE', #36014, #56913, #4577 ) ;
#93864=ADVANCED_FACE ( 'NONE', ( #87525 ), #116977, .T. ) ;
#93865=AXIS2_PLACEMENT_3D ( 'NONE', #87017, #37290, #17625 ) ;
#93866=ORIENTED_EDGE ( 'NONE', *, *, #84737, .F. ) ;
#93867=ORIENTED_EDGE ( 'NONE', *, *, #16112, .T. ) ;
#93868=ORIENTED_EDGE ( 'NONE', *, *, #127978, .T. ) ;
#93869=VERTEX_POINT ( 'NONE', #38457 ) ;
#93870=DIRECTION ( 'NONE',  ( 0.000000000000000000, -0.9999939076577903929, 0.003490651415223739937 ) ) ;
#93871=PLANE ( 'NONE',  #74971 ) ;
#93872=LINE ( 'NONE', #23854, #23808 ) ;
#93873=VERTEX_POINT ( 'NONE', #126822 ) ;
#93874=EDGE_CURVE ( 'NONE', #2220, #61588, #55171, .T. ) ;
#93875=FACE_BOUND ( 'NONE', #21346, .T. ) ;
#93876=ADVANCED_FACE ( 'NONE', ( #77702 ), #44417, .T. ) ;
#93877=CARTESIAN_POINT ( 'NONE',  ( -3.150000000000030109, 12.50000000000000000, -2.446380397790840266 ) ) ;
#93878=LINE ( 'NONE', #14647, #104400 ) ;
#93879=CONICAL_SURFACE ( 'NONE', #95926, 0.1000000000000002554, 0.003490658503988666988 ) ;
#93880=AXIS2_PLACEMENT_3D ( 'NONE', #96809, #37896, #36633 ) ;
#93881=DIRECTION ( 'NONE',  ( 0.000000000000000000, 1.000000000000000000, 0.000000000000000000 ) ) ;
#93882=VECTOR ( 'NONE', #18402, 1000.000000000000000 ) ;
#93883=DIRECTION ( 'NONE',  ( -0.000000000000000000, 1.000000000000000000, -0.000000000000000000 ) ) ;
#93884=DIRECTION ( 'NONE',  ( 0.000000000000000000, -0.000000000000000000, 1.000000000000000000 ) ) ;
#93885=EDGE_CURVE ( 'NONE', #124646, #32011, #118282, .T. ) ;
#93886=DIRECTION ( 'NONE',  ( 0.000000000000000000, 0.000000000000000000, -1.000000000000000000 ) ) ;
#93887=EDGE_CURVE ( 'NONE', #47249, #948, #128345, .T. ) ;
#93888=FACE_OUTER_BOUND ( 'NONE', #80218, .T. ) ;
#93889=CARTESIAN_POINT ( 'NONE',  ( -6.900000000000019007, 12.50000000000000000, -3.983716857408426293 ) ) ;
#93890=EDGE_CURVE ( 'NONE', #38209, #96649, #46318, .T. ) ;
#93891=CARTESIAN_POINT ( 'NONE',  ( 2.949999999999946887, 2.500000000000000000, -6.395190528383301931 ) ) ;
#93892=ADVANCED_FACE ( 'NONE', ( #79025 ), #26687, .T. ) ;
#93893=EDGE_CURVE ( 'NONE', #87565, #77368, #13289, .T. ) ;
#93894=CIRCLE ( 'NONE', #52126, 0.06509327318403745899 ) ;
#93895=CARTESIAN_POINT ( 'NONE',  ( 9.399999999999918643, 2.500000000000000000, 0.4464101615137736623 ) ) ;
#93896=VERTEX_POINT ( 'NONE', #58090 ) ;
#93897=CIRCLE ( 'NONE', #37471, 0.1000000000000002554 ) ;
#93898=ORIENTED_EDGE ( 'NONE', *, *, #116504, .T. ) ;
#93899=VERTEX_POINT ( 'NONE', #46984 ) ;
#93900=ORIENTED_EDGE ( 'NONE', *, *, #13126, .F. ) ;
#93901=EDGE_LOOP ( 'NONE', ( #863, #123052 ) ) ;
#93902=EDGE_LOOP ( 'NONE', ( #40267, #121862, #98357, #37046 ) ) ;
#93903=PLANE ( 'NONE',  #94566 ) ;
#93904=EDGE_LOOP ( 'NONE', ( #58095, #8116 ) ) ;
#93905=ADVANCED_FACE ( 'NONE', ( #106527 ), #44712, .T. ) ;
#93906=EDGE_LOOP ( 'NONE', ( #122018, #98208 ) ) ;
#93907=EDGE_CURVE ( 'NONE', #30951, #72795, #117834, .T. ) ;
#93908=CARTESIAN_POINT ( 'NONE',  ( 12.07106445339097256, -1.499999999999809264, 8.629160868130600903 ) ) ;
#93909=DIRECTION ( 'NONE',  ( -0.000000000000000000, -1.000000000000000000, -0.000000000000000000 ) ) ;
#93910=DIRECTION ( 'NONE',  ( 0.000000000000000000, 1.000000000000000000, 0.000000000000000000 ) ) ;
#93911=AXIS2_PLACEMENT_3D ( 'NONE', #75528, #45459, #125295 ) ;
#93912=ORIENTED_EDGE ( 'NONE', *, *, #113067, .F. ) ;
#93913=LINE ( 'NONE', #97608, #82042 ) ;
#93914=ORIENTED_EDGE ( 'NONE', *, *, #67389, .T. ) ;
#93915=ORIENTED_EDGE ( 'NONE', *, *, #104377, .F. ) ;
#93916=CARTESIAN_POINT ( 'NONE',  ( -5.450000000000019718, 2.500000000000000000, 2.265063509461097357 ) ) ;
#93917=ORIENTED_EDGE ( 'NONE', *, *, #39793, .T. ) ;
#93918=DIRECTION ( 'NONE',  ( 0.000000000000000000, -0.000000000000000000, 1.000000000000000000 ) ) ;
#93919=VERTEX_POINT ( 'NONE', #80950 ) ;
#93920=AXIS2_PLACEMENT_3D ( 'NONE', #93136, #42767, #82678 ) ;
#93921=CARTESIAN_POINT ( 'NONE',  ( -6.250000000000015987, 2.500000000000000000, 5.702370205355745014 ) ) ;
#93922=CARTESIAN_POINT ( 'NONE',  ( -12.89999999999999147, 2.500000000000000000, -4.330127018922198978 ) ) ;
#93923=DIRECTION ( 'NONE',  ( 0.000000000000000000, 0.000000000000000000, -1.000000000000000000 ) ) ;
#93924=LINE ( 'NONE', #44171, #102686 ) ;
#93925=CARTESIAN_POINT ( 'NONE',  ( -13.34999999999999076, 12.50000000000000000, -2.922977105672689202 ) ) ;
#93926=ADVANCED_FACE ( 'NONE', ( #111694 ), #119916, .T. ) ;
#93927=VERTEX_POINT ( 'NONE', #31850 ) ;
#93928=EDGE_CURVE ( 'NONE', #122474, #89282, #71771, .T. ) ;
#93929=CARTESIAN_POINT ( 'NONE',  ( -7.950000000000012612, 2.500000000000000000, -2.065063509461102065 ) ) ;
#93930=ORIENTED_EDGE ( 'NONE', *, *, #68631, .T. ) ;
#93931=CARTESIAN_POINT ( 'NONE',  ( -3.350000000000032507, 2.500000000000000000, -6.395190528383301931 ) ) ;
#93932=EDGE_CURVE ( 'NONE', #65807, #119406, #15144, .T. ) ;
#93933=AXIS2_PLACEMENT_3D ( 'NONE', #77058, #8301, #88806 ) ;
#93934=AXIS2_PLACEMENT_3D ( 'NONE', #14143, #82266, #94637 ) ;
#93935=EDGE_LOOP ( 'NONE', ( #5393, #73846, #67400, #12304 ) ) ;
#93936=DIRECTION ( 'NONE',  ( 0.000000000000000000, 0.000000000000000000, -1.000000000000000000 ) ) ;
#93937=CARTESIAN_POINT ( 'NONE',  ( 8.749999999999953815, 2.500000000000000000, -2.265063509461101798 ) ) ;
#93938=CIRCLE ( 'NONE', #31168, 0.06509327318403745899 ) ;
#93939=DIRECTION ( 'NONE',  ( 0.000000000000000000, 0.000000000000000000, 1.000000000000000000 ) ) ;
#93941=FACE_OUTER_BOUND ( 'NONE', #113574, .T. ) ;
#93942=ORIENTED_EDGE ( 'NONE', *, *, #69098, .F. ) ;
#93943=EDGE_CURVE ( 'NONE', #13400, #125465, #71908, .T. ) ;
#93944=CONICAL_SURFACE ( 'NONE', #87662, 0.09999999999999999167, 0.003490658503988666988 ) ;
#93945=CONICAL_SURFACE ( 'NONE', #18719, 0.09999999999999982514, 0.003490658503988666988 ) ;
#93946=EDGE_CURVE ( 'NONE', #50900, #103695, #123820, .T. ) ;
#93947=DIRECTION ( 'NONE',  ( -0.000000000000000000, 1.000000000000000000, -0.000000000000000000 ) ) ;
#93948=ORIENTED_EDGE ( 'NONE', *, *, #113877, .T. ) ;
#93949=ORIENTED_EDGE ( 'NONE', *, *, #127487, .F. ) ;
#93950=ORIENTED_EDGE ( 'NONE', *, *, #17941, .F. ) ;
#93951=DIRECTION ( 'NONE',  ( 0.000000000000000000, 0.000000000000000000, 1.000000000000000000 ) ) ;
#93954=DIRECTION ( 'NONE',  ( -4.274815082592931898E-19, -0.9999939076577903929, -0.003490651415223739937 ) ) ;
#93955=EDGE_CURVE ( 'NONE', #87480, #6221, #96917, .T. ) ;
#93956=FACE_OUTER_BOUND ( 'NONE', #546, .T. ) ;
#93957=CARTESIAN_POINT ( 'NONE',  ( 12.04999999999990479, 2.500000000000000000, -6.495190528383302464 ) ) ;
#93958=ORIENTED_EDGE ( 'NONE', *, *, #107516, .F. ) ;
#93959=PLANE ( 'NONE',  #119548 ) ;
#93960=AXIS2_PLACEMENT_3D ( 'NONE', #21527, #102023, #12965 ) ;
#93961=AXIS2_PLACEMENT_3D ( 'NONE', #33904, #124864, #73820 ) ;
#93962=ORIENTED_EDGE ( 'NONE', *, *, #87929, .F. ) ;
#93963=CARTESIAN_POINT ( 'NONE',  ( 6.899999999999928413, 12.50000000000000000, -3.983716857408426293 ) ) ;
#93964=DIRECTION ( 'NONE',  ( 0.000000000000000000, 0.000000000000000000, -1.000000000000000000 ) ) ;
#93965=EDGE_CURVE ( 'NONE', #7088, #9874, #4677, .T. ) ;
#93966=DIRECTION ( 'NONE',  ( 0.000000000000000000, 1.000000000000000000, 0.000000000000000000 ) ) ;
#93967=DIRECTION ( 'NONE',  ( -4.274815082592931898E-19, -0.9999939076577903929, -0.003490651415223739937 ) ) ;
#93968=CONICAL_SURFACE ( 'NONE', #125356, 0.09999999999999982514, 0.003490658503988666988 ) ;
#93969=ORIENTED_EDGE ( 'NONE', *, *, #85583, .F. ) ;
#93970=VECTOR ( 'NONE', #110349, 1000.000000000000000 ) ;
#93971=AXIS2_PLACEMENT_3D ( 'NONE', #95526, #56229, #25475 ) ;
#93972=CARTESIAN_POINT ( 'NONE',  ( 12.04999999999990834, 12.50000000000000000, -2.230156782645139391 ) ) ;
#93973=FACE_OUTER_BOUND ( 'NONE', #84796, .T. ) ;
#93974=ORIENTED_EDGE ( 'NONE', *, *, #86570, .T. ) ;
#93975=AXIS2_PLACEMENT_3D ( 'NONE', #16551, #56482, #6719 ) ;
#93976=VERTEX_POINT ( 'NONE', #119562 ) ;
#93978=VECTOR ( 'NONE', #111505, 1000.000000000000000 ) ;
#93980=EDGE_CURVE ( 'NONE', #102949, #35583, #111602, .T. ) ;
#93981=ORIENTED_EDGE ( 'NONE', *, *, #87266, .T. ) ;
#93982=ORIENTED_EDGE ( 'NONE', *, *, #98280, .F. ) ;
#93983=DIRECTION ( 'NONE',  ( -0.000000000000000000, 1.000000000000000000, -0.000000000000000000 ) ) ;
#93984=ORIENTED_EDGE ( 'NONE', *, *, #90635, .T. ) ;
#93985=DIRECTION ( 'NONE',  ( 0.000000000000000000, 1.000000000000000000, 0.000000000000000000 ) ) ;
#93986=FACE_OUTER_BOUND ( 'NONE', #6114, .T. ) ;
#93987=DIRECTION ( 'NONE',  ( 0.000000000000000000, 1.000000000000000000, 0.000000000000000000 ) ) ;
#93988=VERTEX_POINT ( 'NONE', #19428 ) ;
#93989=CARTESIAN_POINT ( 'NONE',  ( 9.799999999999915445, 2.500000000000000000, -4.776537180435977525 ) ) ;
#93990=CARTESIAN_POINT ( 'NONE',  ( -3.300000000000027800, 12.50000000000000000, -4.330127018922201643 ) ) ;
#93991=ORIENTED_EDGE ( 'NONE', *, *, #39993, .F. ) ;
#93992=CIRCLE ( 'NONE', #110703, 0.06509327318403745899 ) ;
#93993=DIRECTION ( 'NONE',  ( -4.274815082592931898E-19, -0.9999939076577903929, -0.003490651415223739937 ) ) ;
#93994=ADVANCED_FACE ( 'NONE', ( #101227 ), #15433, .T. ) ;
#93995=CARTESIAN_POINT ( 'NONE',  ( -9.150000000000011013, 12.50000000000000000, -5.737276932171707422 ) ) ;
#93996=EDGE_LOOP ( 'NONE', ( #116008, #50035 ) ) ;
#93997=VERTEX_POINT ( 'NONE', #12179 ) ;
#93998=VERTEX_POINT ( 'NONE', #109763 ) ;
#93999=DIRECTION ( 'NONE',  ( 0.000000000000000000, -0.9999939076577903929, 0.003490651415223739937 ) ) ;
#94000=CARTESIAN_POINT ( 'NONE',  ( 3.749999999999940492, 2.500000000000000000, 2.757883832488649656 ) ) ;
#94001=CARTESIAN_POINT ( 'NONE',  ( 4.349999999999940137, 2.500000000000000000, -6.741600689897078169 ) ) ;
#94002=FACE_BOUND ( 'NONE', #95632, .T. ) ;
#94003=ORIENTED_EDGE ( 'NONE', *, *, #66722, .T. ) ;
#94005=CARTESIAN_POINT ( 'NONE',  ( 6.249999999999930722, 2.500000000000000000, 1.372243186433545370 ) ) ;
#94006=DIRECTION ( 'NONE',  ( -0.000000000000000000, 1.000000000000000000, -0.000000000000000000 ) ) ;
#94007=LINE ( 'NONE', #42340, #54742 ) ;
#94008=CARTESIAN_POINT ( 'NONE',  ( -1.650000000000034328, 2.500000000000000000, -2.957883832488653830 ) ) ;
#94009=CIRCLE ( 'NONE', #85691, 0.06509327318403745899 ) ;
#94010=FACE_OUTER_BOUND ( 'NONE', #127409, .T. ) ;
#94011=CARTESIAN_POINT ( 'NONE',  ( 0.5999999999999621192, 2.500000000000000000, 0.3464101615137758494 ) ) ;
#94012=ADVANCED_FACE ( 'NONE', ( #59396 ), #66975, .T. ) ;
#94013=CIRCLE ( 'NONE', #68976, 0.09999999999999982514 ) ;
#94014=CIRCLE ( 'NONE', #54313, 0.06509327318403745899 ) ;
#94015=VERTEX_POINT ( 'NONE', #112975 ) ;
#94016=ORIENTED_EDGE ( 'NONE', *, *, #129252, .F. ) ;
#94017=EDGE_LOOP ( 'NONE', ( #110477, #57015, #106234, #8227 ) ) ;
#94018=VERTEX_POINT ( 'NONE', #102512 ) ;
#94019=ORIENTED_EDGE ( 'NONE', *, *, #101498, .T. ) ;
#94020=LINE ( 'NONE', #44268, #61035 ) ;
#94021=CIRCLE ( 'NONE', #108598, 0.06509327318403741736 ) ;
#94022=FACE_OUTER_BOUND ( 'NONE', #29532, .T. ) ;
#94023=ORIENTED_EDGE ( 'NONE', *, *, #46585, .F. ) ;
#94024=FACE_BOUND ( 'NONE', #107945, .T. ) ;
#94025=FACE_OUTER_BOUND ( 'NONE', #53465, .T. ) ;
#94026=EDGE_CURVE ( 'NONE', #13985, #106765, #112338, .T. ) ;
#94027=AXIS2_PLACEMENT_3D ( 'NONE', #53237, #33597, #43431 ) ;
#94028=CIRCLE ( 'NONE', #56366, 0.1000000000000002554 ) ;
#94029=VERTEX_POINT ( 'NONE', #104444 ) ;
#94030=EDGE_CURVE ( 'NONE', #117860, #90471, #54059, .T. ) ;
#94031=LINE ( 'NONE', #104491, #83018 ) ;
#94032=ADVANCED_FACE ( 'NONE', ( #63880 ), #84149, .T. ) ;
#94033=DIRECTION ( 'NONE',  ( 0.000000000000000000, 1.000000000000000000, 0.000000000000000000 ) ) ;
#94034=EDGE_CURVE ( 'NONE', #84904, #91963, #52763, .T. ) ;
#94035=CARTESIAN_POINT ( 'NONE',  ( 4.549999999999939426, 2.500000000000000000, -2.065063509461102065 ) ) ;
#94036=ADVANCED_FACE ( 'NONE', ( #23294 ), #103189, .T. ) ;
#94037=ORIENTED_EDGE ( 'NONE', *, *, #22672, .F. ) ;
#94038=DIRECTION ( 'NONE',  ( -0.000000000000000000, 1.000000000000000000, -0.000000000000000000 ) ) ;
#94039=ORIENTED_EDGE ( 'NONE', *, *, #70579, .T. ) ;
#94040=EDGE_CURVE ( 'NONE', #2601, #92856, #4936, .T. ) ;
#94041=ORIENTED_EDGE ( 'NONE', *, *, #77810, .T. ) ;
#94042=VERTEX_POINT ( 'NONE', #35081 ) ;
#94043=CARTESIAN_POINT ( 'NONE',  ( 10.39999999999991154, 12.50000000000000000, 4.957854068765711553 ) ) ;
#94044=LINE ( 'NONE', #4342, #98572 ) ;
#94045=DIRECTION ( 'NONE',  ( 0.000000000000000000, 1.000000000000000000, 0.000000000000000000 ) ) ;
#94046=EDGE_LOOP ( 'NONE', ( #7295, #2284 ) ) ;
#94047=ADVANCED_FACE ( 'NONE', ( #74988 ), #114897, .T. ) ;
#94048=CARTESIAN_POINT ( 'NONE',  ( -9.150000000000009237, 2.500000000000000000, 2.757883832488649656 ) ) ;
#94049=EDGE_CURVE ( 'NONE', #109495, #92601, #80220, .T. ) ;
#94050=AXIS2_PLACEMENT_3D ( 'NONE', #32982, #102983, #63717 ) ;
#94051=DIRECTION ( 'NONE',  ( 0.000000000000000000, 0.000000000000000000, 1.000000000000000000 ) ) ;
#94052=EDGE_CURVE ( 'NONE', #122843, #19850, #33962, .T. ) ;
#94053=AXIS2_PLACEMENT_3D ( 'NONE', #15300, #106283, #4193 ) ;
#94056=EDGE_LOOP ( 'NONE', ( #121170, #2978 ) ) ;
#94057=DIRECTION ( 'NONE',  ( 0.000000000000000000, -0.000000000000000000, 1.000000000000000000 ) ) ;
#94058=ADVANCED_FACE ( 'NONE', ( #3033 ), #92696, .T. ) ;
#94059=ORIENTED_EDGE ( 'NONE', *, *, #60104, .T. ) ;
#94060=DIRECTION ( 'NONE',  ( 0.000000000000000000, 0.000000000000000000, -1.000000000000000000 ) ) ;
#94061=CIRCLE ( 'NONE', #62681, 0.1000000000000002554 ) ;
#94062=ORIENTED_EDGE ( 'NONE', *, *, #105328, .T. ) ;
#94063=ORIENTED_EDGE ( 'NONE', *, *, #116502, .F. ) ;
#94064=DIRECTION ( 'NONE',  ( 0.000000000000000000, 1.000000000000000000, 0.000000000000000000 ) ) ;
#94066=DIRECTION ( 'NONE',  ( -0.000000000000000000, 1.000000000000000000, -0.000000000000000000 ) ) ;
#94067=CARTESIAN_POINT ( 'NONE',  ( -11.64999999999999680, 2.500000000000000000, -2.165063509461097713 ) ) ;
#94068=CARTESIAN_POINT ( 'NONE',  ( -9.150000000000009237, 2.500000000000000000, -7.288010851410849256 ) ) ;
#94069=CONICAL_SURFACE ( 'NONE', #108729, 0.09999999999999982514, 0.003490658503988666988 ) ;
#94070=EDGE_LOOP ( 'NONE', ( #26397, #21378 ) ) ;
#94071=VERTEX_POINT ( 'NONE', #13473 ) ;
#94072=CIRCLE ( 'NONE', #39727, 0.09999999999999982514 ) ;
#94073=DIRECTION ( 'NONE',  ( 0.000000000000000000, -0.000000000000000000, 1.000000000000000000 ) ) ;
#94074=AXIS2_PLACEMENT_3D ( 'NONE', #75314, #43941, #84503 ) ;
#94075=DIRECTION ( 'NONE',  ( -0.000000000000000000, 1.000000000000000000, -0.000000000000000000 ) ) ;
#94076=CARTESIAN_POINT ( 'NONE',  ( -7.300000000000014921, 2.500000000000000000, 4.576537180435972019 ) ) ;
#94077=ORIENTED_EDGE ( 'NONE', *, *, #55319, .T. ) ;
#94078=ORIENTED_EDGE ( 'NONE', *, *, #45290, .F. ) ;
#94079=AXIS2_PLACEMENT_3D ( 'NONE', #87758, #6594, #18381 ) ;
#94080=CARTESIAN_POINT ( 'NONE',  ( 7.499999999999923617, 2.500000000000000000, 0.5928203230275495006 ) ) ;
#94081=CIRCLE ( 'NONE', #102402, 0.06509327318403745899 ) ;
#94082=ORIENTED_EDGE ( 'NONE', *, *, #36838, .T. ) ;
#94083=CARTESIAN_POINT ( 'NONE',  ( -1.650000000000035660, 2.500000000000000000, 7.188010851410848723 ) ) ;
#94084=FACE_OUTER_BOUND ( 'NONE', #17073, .T. ) ;
#94085=VERTEX_POINT ( 'NONE', #107002 ) ;
#94086=LINE ( 'NONE', #23397, #98331 ) ;
#94087=DIRECTION ( 'NONE',  ( 0.000000000000000000, 0.000000000000000000, -1.000000000000000000 ) ) ;
#94088=AXIS2_PLACEMENT_3D ( 'NONE', #123769, #123150, #33495 ) ;
#94089=DIRECTION ( 'NONE',  ( 0.000000000000000000, 0.000000000000000000, 1.000000000000000000 ) ) ;
#94090=DIRECTION ( 'NONE',  ( 0.000000000000000000, -0.000000000000000000, 1.000000000000000000 ) ) ;
#94091=ORIENTED_EDGE ( 'NONE', *, *, #116484, .T. ) ;
#94092=EDGE_CURVE ( 'NONE', #122396, #51312, #47463, .T. ) ;
#94093=FACE_OUTER_BOUND ( 'NONE', #17131, .T. ) ;
#94094=LINE ( 'NONE', #83640, #81151 ) ;
#94095=EDGE_CURVE ( 'NONE', #12403, #1184, #90668, .T. ) ;
#94096=ORIENTED_EDGE ( 'NONE', *, *, #32349, .F. ) ;
#94097=VERTEX_POINT ( 'NONE', #115534 ) ;
#94099=DIRECTION ( 'NONE',  ( -0.000000000000000000, 1.000000000000000000, -0.000000000000000000 ) ) ;
#94100=DIRECTION ( 'NONE',  ( 0.000000000000000000, 0.000000000000000000, 1.000000000000000000 ) ) ;
#94101=CARTESIAN_POINT ( 'NONE',  ( 6.699999999999928235, 2.500000000000000000, -0.1000000000000022815 ) ) ;
#94102=EDGE_CURVE ( 'NONE', #70406, #25375, #84407, .T. ) ;
#94103=FACE_OUTER_BOUND ( 'NONE', #126968, .T. ) ;
#94104=DIRECTION ( 'NONE',  ( -0.000000000000000000, -1.000000000000000000, -0.000000000000000000 ) ) ;
#94105=CARTESIAN_POINT ( 'NONE',  ( -10.20000000000000284, 12.50000000000000000, 3.918623584224383727 ) ) ;
#94106=LINE ( 'NONE', #33278, #92991 ) ;
#94107=CARTESIAN_POINT ( 'NONE',  ( -6.900000000000015454, 12.50000000000000000, 4.676537180435972552 ) ) ;
#94108=CARTESIAN_POINT ( 'NONE',  ( -4.350000000000023626, 12.50000000000000000, 6.148780366869520897 ) ) ;
#94109=AXIS2_PLACEMENT_3D ( 'NONE', #31789, #101171, #30518 ) ;
#94110=CARTESIAN_POINT ( 'NONE',  ( 2.899999999999946620, 2.500000000000000000, -0.6928203230275542523 ) ) ;
#94111=ORIENTED_EDGE ( 'NONE', *, *, #87154, .F. ) ;
#94112=ORIENTED_EDGE ( 'NONE', *, *, #62731, .T. ) ;
#94113=CIRCLE ( 'NONE', #37684, 0.1000000000000002554 ) ;
#94114=AXIS2_PLACEMENT_3D ( 'NONE', #83401, #84018, #61833 ) ;
#94115=EDGE_LOOP ( 'NONE', ( #18505, #59244 ) ) ;
#94116=EDGE_LOOP ( 'NONE', ( #108869, #63991 ) ) ;
#94117=PLANE ( 'NONE',  #12326 ) ;
#94118=DIRECTION ( 'NONE',  ( 0.000000000000000000, 1.000000000000000000, 0.000000000000000000 ) ) ;
#94119=DIRECTION ( 'NONE',  ( -4.274815082592931898E-19, -0.9999939076577903929, -0.003490651415223739937 ) ) ;
#94120=CIRCLE ( 'NONE', #110740, 0.06509327318403745899 ) ;
#94121=ORIENTED_EDGE ( 'NONE', *, *, #5673, .T. ) ;
#94122=FACE_OUTER_BOUND ( 'NONE', #55719, .T. ) ;
#94123=CARTESIAN_POINT ( 'NONE',  ( -4.400000000000028777, 12.50000000000000000, -3.983716857408426293 ) ) ;
#94124=CARTESIAN_POINT ( 'NONE',  ( -1.900000000000035438, 12.50000000000000000, 3.918623584224382839 ) ) ;
#94125=VERTEX_POINT ( 'NONE', #117448 ) ;
#94126=DIRECTION ( 'NONE',  ( 0.000000000000000000, 1.000000000000000000, 0.000000000000000000 ) ) ;
#94127=DIRECTION ( 'NONE',  ( -1.000000000000000000, -0.000000000000000000, -0.000000000000000000 ) ) ;
#94129=VERTEX_POINT ( 'NONE', #75610 ) ;
#94130=EDGE_LOOP ( 'NONE', ( #41407, #19606, #101723, #17767 ) ) ;
#94132=LINE ( 'NONE', #55504, #51043 ) ;
#94133=CARTESIAN_POINT ( 'NONE',  ( 7.299999999999926104, 2.500000000000000000, 4.776537180435972196 ) ) ;
#94134=CARTESIAN_POINT ( 'NONE',  ( 6.249999999999967137, 12.50000000000000000, 6.495190528383297135 ) ) ;
#94135=DIRECTION ( 'NONE',  ( 0.000000000000000000, -0.9999939076577903929, 0.003490651415223739937 ) ) ;
#94136=AXIS2_PLACEMENT_3D ( 'NONE', #18889, #17597, #127567 ) ;
#94138=ORIENTED_EDGE ( 'NONE', *, *, #115148, .F. ) ;
#94139=CIRCLE ( 'NONE', #20981, 0.06509327318403741736 ) ;
#94140=PLANE ( 'NONE',  #125449 ) ;
#94141=EDGE_CURVE ( 'NONE', #79210, #113203, #67738, .T. ) ;
#94143=DIRECTION ( 'NONE',  ( 0.000000000000000000, 1.000000000000000000, 0.000000000000000000 ) ) ;
#94144=CARTESIAN_POINT ( 'NONE',  ( 12.64862127202683872, -1.499999999999935607, -8.430718248283369576 ) ) ;
#94145=CARTESIAN_POINT ( 'NONE',  ( 11.24999999999990585, 2.500000000000000000, -5.902370205355750521 ) ) ;
#94146=CARTESIAN_POINT ( 'NONE',  ( 20.37025966759669515, -0.6621301594403563584, 4.188616773932332116 ) ) ;
#94147=EDGE_CURVE ( 'NONE', #66442, #60131, #77853, .T. ) ;
#94148=AXIS2_PLACEMENT_3D ( 'NONE', #60823, #50352, #90254 ) ;
#94149=ORIENTED_EDGE ( 'NONE', *, *, #10657, .F. ) ;
#94150=ORIENTED_EDGE ( 'NONE', *, *, #97865, .F. ) ;
#94151=ORIENTED_EDGE ( 'NONE', *, *, #418, .F. ) ;
#94152=DIRECTION ( 'NONE',  ( 0.000000000000000000, 0.000000000000000000, -1.000000000000000000 ) ) ;
#94153=CARTESIAN_POINT ( 'NONE',  ( -6.650000000000018119, 2.500000000000000000, -7.188010851410854052 ) ) ;
#94154=EDGE_CURVE ( 'NONE', #89533, #35730, #37003, .T. ) ;
#94155=LINE ( 'NONE', #86907, #25200 ) ;
#94156=FACE_BOUND ( 'NONE', #100777, .T. ) ;
#94157=DIRECTION ( 'NONE',  ( 0.000000000000000000, 0.000000000000000000, 1.000000000000000000 ) ) ;
#94158=CARTESIAN_POINT ( 'NONE',  ( -13.34999999999999076, 2.500000000000000000, 2.857883832488652853 ) ) ;
#94159=DIRECTION ( 'NONE',  ( -0.000000000000000000, 1.000000000000000000, -0.000000000000000000 ) ) ;
#94160=AXIS2_PLACEMENT_3D ( 'NONE', #54365, #2671, #101541 ) ;
#94161=CIRCLE ( 'NONE', #92095, 0.06509327318403745899 ) ;
#94163=CARTESIAN_POINT ( 'NONE',  ( 11.04999999999991012, 2.500000000000000000, -1.918653347947326004 ) ) ;
#94165=DIRECTION ( 'NONE',  ( -0.000000000000000000, 1.000000000000000000, -0.000000000000000000 ) ) ;
#94166=VERTEX_POINT ( 'NONE', #6222 ) ;
#94167=CIRCLE ( 'NONE', #46060, 0.06509327318403745899 ) ;
#94168=CARTESIAN_POINT ( 'NONE',  ( 6.049999999999935874, 2.500000000000000000, -6.841600689897077814 ) ) ;
#94169=EDGE_CURVE ( 'NONE', #89954, #19824, #37654, .T. ) ;
#94170=ORIENTED_EDGE ( 'NONE', *, *, #50888, .T. ) ;
#94171=AXIS2_PLACEMENT_3D ( 'NONE', #70667, #60232, #121694 ) ;
#94172=ORIENTED_EDGE ( 'NONE', *, *, #20782, .F. ) ;
#94173=ORIENTED_EDGE ( 'NONE', *, *, #117200, .F. ) ;
#94174=ORIENTED_EDGE ( 'NONE', *, *, #98910, .F. ) ;
#94175=DIRECTION ( 'NONE',  ( 0.000000000000000000, -0.000000000000000000, 1.000000000000000000 ) ) ;
#94176=FACE_BOUND ( 'NONE', #61022, .T. ) ;
#94177=DIRECTION ( 'NONE',  ( 0.000000000000000000, 0.000000000000000000, 1.000000000000000000 ) ) ;
#94178=ADVANCED_FACE ( 'NONE', ( #76921 ), #28474, .T. ) ;
#94179=ORIENTED_EDGE ( 'NONE', *, *, #20201, .T. ) ;
#94180=EDGE_CURVE ( 'NONE', #101722, #87021, #27774, .T. ) ;
#94181=DIRECTION ( 'NONE',  ( 0.000000000000000000, 0.000000000000000000, 1.000000000000000000 ) ) ;
#94182=ADVANCED_FACE ( 'NONE', ( #107673 ), #17991, .T. ) ;
#94183=LINE ( 'NONE', #4485, #123017 ) ;
#94185=ADVANCED_FACE ( 'NONE', ( #118127 ), #108307, .T. ) ;
#94186=ORIENTED_EDGE ( 'NONE', *, *, #95685, .T. ) ;
#94187=CARTESIAN_POINT ( 'NONE',  ( -8.550000000000013145, 2.500000000000000000, -1.818653347947326138 ) ) ;
#94188=DIRECTION ( 'NONE',  ( 0.000000000000000000, -0.9999939076577903929, 0.003490651415223739937 ) ) ;
#94189=EDGE_CURVE ( 'NONE', #50586, #35208, #57012, .T. ) ;
#94192=AXIS2_PLACEMENT_3D ( 'NONE', #90551, #70283, #61099 ) ;
#94193=CARTESIAN_POINT ( 'NONE',  ( 6.449999999999930012, 2.500000000000000000, -1.818653347947326138 ) ) ;
#94194=AXIS2_PLACEMENT_3D ( 'NONE', #8258, #78321, #39053 ) ;
#94195=EDGE_CURVE ( 'NONE', #117091, #54998, #34051, .T. ) ;
#94196=CARTESIAN_POINT ( 'NONE',  ( -3.750000000000031086, 2.500000000000000000, -5.802370205355749988 ) ) ;
#94197=ADVANCED_FACE ( 'NONE', ( #56612 ), #21526, .T. ) ;
#94198=EDGE_LOOP ( 'NONE', ( #2917, #1175, #45574, #112492 ) ) ;
#94199=DIRECTION ( 'NONE',  ( 0.000000000000000000, 0.000000000000000000, -1.000000000000000000 ) ) ;
#94200=AXIS2_PLACEMENT_3D ( 'NONE', #40715, #80628, #100263 ) ;
#94201=ADVANCED_FACE ( 'NONE', ( #89955 ), #118777, .T. ) ;
#94202=CARTESIAN_POINT ( 'NONE',  ( -1.050000000000037792, 12.50000000000000000, 1.818653347947321475 ) ) ;
#94203=FACE_OUTER_BOUND ( 'NONE', #21985, .T. ) ;
#94204=ORIENTED_EDGE ( 'NONE', *, *, #82123, .T. ) ;
#94205=ORIENTED_EDGE ( 'NONE', *, *, #101456, .F. ) ;
#94206=EDGE_CURVE ( 'NONE', #48754, #67150, #13095, .T. ) ;
#94207=DIRECTION ( 'NONE',  ( 0.000000000000000000, -0.9999939076577903929, 0.003490651415223739937 ) ) ;
#94208=ADVANCED_FACE ( 'NONE', ( #29753 ), #119714, .T. ) ;
#94209=ORIENTED_EDGE ( 'NONE', *, *, #52198, .T. ) ;
#94210=CARTESIAN_POINT ( 'NONE',  ( -14.34999999999998543, 2.500000000000000000, -1.918653347947323784 ) ) ;
#94211=CARTESIAN_POINT ( 'NONE',  ( 8.099999999999923261, 2.500000000000000000, -3.983716857408426293 ) ) ;
#94212=ORIENTED_EDGE ( 'NONE', *, *, #50563, .T. ) ;
#94213=DIRECTION ( 'NONE',  ( 0.000000000000000000, 0.000000000000000000, 1.000000000000000000 ) ) ;
#94214=CARTESIAN_POINT ( 'NONE',  ( -6.250000000000017764, 12.50000000000000000, 2.857883832488649301 ) ) ;
#94215=LINE ( 'NONE', #103400, #102967 ) ;
#94216=DIRECTION ( 'NONE',  ( -0.000000000000000000, 1.000000000000000000, -0.000000000000000000 ) ) ;
#94217=DIRECTION ( 'NONE',  ( 0.000000000000000000, 1.000000000000000000, 0.000000000000000000 ) ) ;
#94218=VERTEX_POINT ( 'NONE', #129273 ) ;
#94220=CARTESIAN_POINT ( 'NONE',  ( 11.84999999999990727, 2.500000000000000000, 6.841600689897072485 ) ) ;
#94221=DIRECTION ( 'NONE',  ( 0.000000000000000000, -0.9999939076577903929, 0.003490651415223739937 ) ) ;
#94222=CARTESIAN_POINT ( 'NONE',  ( 5.199999999999935341, 2.500000000000000000, -4.083716857408426826 ) ) ;
#94223=ORIENTED_EDGE ( 'NONE', *, *, #80567, .F. ) ;
#94224=ORIENTED_EDGE ( 'NONE', *, *, #28582, .F. ) ;
#94225=EDGE_LOOP ( 'NONE', ( #5095, #15331 ) ) ;
#94226=CARTESIAN_POINT ( 'NONE',  ( -2.499999999999996003, 2.500000000000000000, 0.09999999999999772959 ) ) ;
#94227=VECTOR ( 'NONE', #7968, 1000.000000000000000 ) ;
#94228=DIRECTION ( 'NONE',  ( 0.000000000000000000, -0.000000000000000000, 1.000000000000000000 ) ) ;
#94229=AXIS2_PLACEMENT_3D ( 'NONE', #18740, #119513, #39059 ) ;
#94230=DIRECTION ( 'NONE',  ( 0.000000000000000000, 0.000000000000000000, 1.000000000000000000 ) ) ;
#94232=DIRECTION ( 'NONE',  ( 0.000000000000000000, -0.9999939076577903929, 0.003490651415223739937 ) ) ;
#94233=CARTESIAN_POINT ( 'NONE',  ( 8.549999999999922551, 2.500000000000000000, 2.411473670974873862 ) ) ;
#94234=CARTESIAN_POINT ( 'NONE',  ( 0.5999999999999547917, 2.500000000000000000, 3.883716857408420431 ) ) ;
#94235=DIRECTION ( 'NONE',  ( 0.000000000000000000, 0.000000000000000000, 1.000000000000000000 ) ) ;
#94236=CARTESIAN_POINT ( 'NONE',  ( -4.400000000000025224, 12.50000000000000000, 0.3464101615137735735 ) ) ;
#94237=DIRECTION ( 'NONE',  ( 0.000000000000000000, -0.000000000000000000, 1.000000000000000000 ) ) ;
#94238=CIRCLE ( 'NONE', #4327, 0.1000000000000002554 ) ;
#94239=VECTOR ( 'NONE', #116618, 1000.000000000000000 ) ;
#94240=EDGE_LOOP ( 'NONE', ( #121485, #74437, #47300, #40376 ) ) ;
#94241=EDGE_CURVE ( 'NONE', #51418, #117845, #107197, .T. ) ;
#94242=EDGE_CURVE ( 'NONE', #31947, #24001, #101075, .T. ) ;
#94243=CARTESIAN_POINT ( 'NONE',  ( 12.09999999999990550, 12.50000000000000000, 4.265033745738159077 ) ) ;
#94244=EDGE_LOOP ( 'NONE', ( #31697, #101111 ) ) ;
#94245=EDGE_LOOP ( 'NONE', ( #117923, #52137 ) ) ;
#94246=DIRECTION ( 'NONE',  ( 0.000000000000000000, -0.9999939076577903929, 0.003490651415223739937 ) ) ;
#94247=DIRECTION ( 'NONE',  ( 0.000000000000000000, 1.000000000000000000, 0.000000000000000000 ) ) ;
#94248=CARTESIAN_POINT ( 'NONE',  ( -8.100000000000010303, 2.500000000000000000, 3.883716857408421319 ) ) ;
#94249=AXIS2_PLACEMENT_3D ( 'NONE', #73852, #33306, #43135 ) ;
#94250=DIRECTION ( 'NONE',  ( -0.000000000000000000, -1.000000000000000000, -0.000000000000000000 ) ) ;
#94251=CIRCLE ( 'NONE', #48380, 0.09999999999999999167 ) ;
#94252=CARTESIAN_POINT ( 'NONE',  ( -5.850000000000022737, 2.500000000000000000, -2.165063509461101710 ) ) ;
#94253=DIRECTION ( 'NONE',  ( 0.000000000000000000, -0.9999939076577903929, 0.003490651415223739937 ) ) ;
#94254=CARTESIAN_POINT ( 'NONE',  ( -12.89999999999999147, 2.500000000000000000, 5.122947341949749323 ) ) ;
#94255=ORIENTED_EDGE ( 'NONE', *, *, #977, .T. ) ;
#94256=DIRECTION ( 'NONE',  ( 0.000000000000000000, 0.000000000000000000, -1.000000000000000000 ) ) ;
#94257=AXIS2_PLACEMENT_3D ( 'NONE', #128136, #77720, #120253 ) ;
#94258=DIRECTION ( 'NONE',  ( -0.000000000000000000, 1.000000000000000000, -0.000000000000000000 ) ) ;
#94259=EDGE_LOOP ( 'NONE', ( #9604, #62465, #52299, #55798 ) ) ;
#94260=ORIENTED_EDGE ( 'NONE', *, *, #110440, .F. ) ;
#94261=AXIS2_PLACEMENT_3D ( 'NONE', #31099, #61842, #31723 ) ;
#94262=VERTEX_POINT ( 'NONE', #19943 ) ;
#94264=CARTESIAN_POINT ( 'NONE',  ( -11.64999999999999680, 2.500000000000000000, -2.957883832488649833 ) ) ;
#94265=CARTESIAN_POINT ( 'NONE',  ( -11.05000000000000249, 2.500000000000000000, -1.718653347947322052 ) ) ;
#94266=DIRECTION ( 'NONE',  ( -0.000000000000000000, 1.000000000000000000, -0.000000000000000000 ) ) ;
#94267=DIRECTION ( 'NONE',  ( -0.000000000000000000, -1.000000000000000000, -0.000000000000000000 ) ) ;
#94268=DIRECTION ( 'NONE',  ( 0.000000000000000000, 0.000000000000000000, -1.000000000000000000 ) ) ;
#94269=ORIENTED_EDGE ( 'NONE', *, *, #105933, .F. ) ;
#94270=CARTESIAN_POINT ( 'NONE',  ( 26.76176527441709396, -1.073658815337092731, 4.445806700577109360 ) ) ;
#94271=DIRECTION ( 'NONE',  ( 0.000000000000000000, -0.9999939076577903929, 0.003490651415223739937 ) ) ;
#94272=DIRECTION ( 'NONE',  ( 0.000000000000000000, -0.000000000000000000, 1.000000000000000000 ) ) ;
#94273=EDGE_CURVE ( 'NONE', #97573, #48757, #111384, .T. ) ;
#94274=EDGE_LOOP ( 'NONE', ( #81948, #74128, #4539, #92318 ) ) ;
#94276=ORIENTED_EDGE ( 'NONE', *, *, #35722, .F. ) ;
#94277=CONICAL_SURFACE ( 'NONE', #69227, 0.09999999999999982514, 0.003490658503988666988 ) ;
#94278=DIRECTION ( 'NONE',  ( 0.000000000000000000, 0.000000000000000000, -1.000000000000000000 ) ) ;
#94279=CIRCLE ( 'NONE', #110907, 0.1000000000000002554 ) ;
#94280=CONICAL_SURFACE ( 'NONE', #85950, 0.1000000000000002554, 0.003490658503988666988 ) ;
#94281=CARTESIAN_POINT ( 'NONE',  ( 1.449999999999949551, 12.50000000000000000, 6.841600689897072485 ) ) ;
#94282=CARTESIAN_POINT ( 'NONE',  ( 1.899999999999951283, 2.500000000000000000, -4.083716857408426826 ) ) ;
#94283=AXIS2_PLACEMENT_3D ( 'NONE', #80884, #11485, #71694 ) ;
#94284=EDGE_CURVE ( 'NONE', #31101, #20569, #48623, .T. ) ;
#94285=ORIENTED_EDGE ( 'NONE', *, *, #80285, .F. ) ;
#94286=DIRECTION ( 'NONE',  ( -0.000000000000000000, 1.000000000000000000, -0.000000000000000000 ) ) ;
#94287=CARTESIAN_POINT ( 'NONE',  ( -9.999999999999969802, 2.500000000000000000, -2.276824562219559311E-15 ) ) ;
#94289=ADVANCED_FACE ( 'NONE', ( #99790 ), #77952, .T. ) ;
#94290=CARTESIAN_POINT ( 'NONE',  ( -9.600000000000006750, 2.500000000000000000, 3.737306695894644371 ) ) ;
#94291=FACE_OUTER_BOUND ( 'NONE', #64442, .T. ) ;
#94292=ORIENTED_EDGE ( 'NONE', *, *, #92511, .T. ) ;
#94293=VERTEX_POINT ( 'NONE', #71607 ) ;
#94294=ADVANCED_FACE ( 'NONE', ( #29129 ), #54966, .T. ) ;
#94295=FACE_OUTER_BOUND ( 'NONE', #15346, .T. ) ;
#94296=PLANE ( 'NONE',  #79100 ) ;
#94297=CARTESIAN_POINT ( 'NONE',  ( -0.4000000000000392131, 2.500000000000000000, -5.122947341949753763 ) ) ;
#94298=CARTESIAN_POINT ( 'NONE',  ( -12.89999999999999147, 12.50000000000000000, -5.022947341949751454 ) ) ;
#94299=CARTESIAN_POINT ( 'NONE',  ( -3.350000000000028511, 2.500000000000000000, 2.757883832488649656 ) ) ;
#94301=CIRCLE ( 'NONE', #125599, 0.06509327318403745899 ) ;
#94302=ORIENTED_EDGE ( 'NONE', *, *, #59324, .T. ) ;
#94303=DIRECTION ( 'NONE',  ( -0.000000000000000000, -1.000000000000000000, -0.000000000000000000 ) ) ;
#94304=FACE_OUTER_BOUND ( 'NONE', #35512, .T. ) ;
#94305=DIRECTION ( 'NONE',  ( 0.000000000000000000, -0.9999939076577903929, 0.003490651415223739937 ) ) ;
#94307=ORIENTED_EDGE ( 'NONE', *, *, #93468, .T. ) ;
#94308=AXIS2_PLACEMENT_3D ( 'NONE', #94917, #45184, #3314 ) ;
#94309=DIRECTION ( 'NONE',  ( 0.000000000000000000, 1.000000000000000000, 0.000000000000000000 ) ) ;
#94310=VECTOR ( 'NONE', #55298, 1000.000000000000000 ) ;
#94311=CARTESIAN_POINT ( 'NONE',  ( 8.149999999999920419, 2.500000000000000000, 6.048780366869521252 ) ) ;
#94312=VERTEX_POINT ( 'NONE', #39605 ) ;
#94313=DIRECTION ( 'NONE',  ( 0.000000000000000000, 1.000000000000000000, 0.000000000000000000 ) ) ;
#94314=ORIENTED_EDGE ( 'NONE', *, *, #124902, .T. ) ;
#94315=CIRCLE ( 'NONE', #44158, 0.06509327318403745899 ) ;
#94316=CARTESIAN_POINT ( 'NONE',  ( 13.74999999999993427, 12.50000000000000000, 2.099970236277060032 ) ) ;
#94317=EDGE_CURVE ( 'NONE', #72203, #20272, #80010, .T. ) ;
#94318=VERTEX_POINT ( 'NONE', #10119 ) ;
#94319=DIRECTION ( 'NONE',  ( 0.000000000000000000, 1.000000000000000000, 0.000000000000000000 ) ) ;
#94320=CARTESIAN_POINT ( 'NONE',  ( -8.550000000000007816, 2.500000000000000000, 6.148780366869520009 ) ) ;
#94321=ORIENTED_EDGE ( 'NONE', *, *, #65790, .T. ) ;
#94322=ORIENTED_EDGE ( 'NONE', *, *, #30085, .F. ) ;
#94323=ADVANCED_FACE ( 'NONE', ( #90600 ), #88405, .T. ) ;
#94325=EDGE_CURVE ( 'NONE', #37140, #49253, #15236, .T. ) ;
#94326=AXIS2_PLACEMENT_3D ( 'NONE', #108459, #7672, #109092 ) ;
#94328=CARTESIAN_POINT ( 'NONE',  ( -5.650000000000019895, 12.50000000000000000, 6.148780366869520009 ) ) ;
#94329=CARTESIAN_POINT ( 'NONE',  ( -11.05000000000000249, 2.500000000000000000, -6.248780366869523206 ) ) ;
#94330=CIRCLE ( 'NONE', #40067, 0.06509327318403745899 ) ;
#94331=DIRECTION ( 'NONE',  ( -4.274815082592931898E-19, -0.9999939076577903929, -0.003490651415223739937 ) ) ;
#94332=ADVANCED_FACE ( 'NONE', ( #31694 ), #42369, .T. ) ;
#94333=EDGE_CURVE ( 'NONE', #69856, #108500, #105136, .T. ) ;
#94334=CARTESIAN_POINT ( 'NONE',  ( 1.649999999999951505, 12.50000000000000000, -1.472243186433550122 ) ) ;
#94335=CARTESIAN_POINT ( 'NONE',  ( 7.949999999999922018, 2.500000000000000000, 6.395190528383296602 ) ) ;
#94336=ADVANCED_FACE ( 'NONE', ( #69022 ), #128630, .T. ) ;
#94337=AXIS2_PLACEMENT_3D ( 'NONE', #32530, #62625, #61329 ) ;
#94338=EDGE_CURVE ( 'NONE', #60021, #52226, #113460, .T. ) ;
#94339=ORIENTED_EDGE ( 'NONE', *, *, #52520, .F. ) ;
#94340=ORIENTED_EDGE ( 'NONE', *, *, #123160, .T. ) ;
#94341=CARTESIAN_POINT ( 'NONE',  ( 0.3999999999999555023, 12.50000000000000000, 4.395220292106234439 ) ) ;
#94342=EDGE_CURVE ( 'NONE', #58914, #5985, #2631, .T. ) ;
#94343=CIRCLE ( 'NONE', #60906, 0.06509327318403745899 ) ;
#94344=CIRCLE ( 'NONE', #27442, 0.06509327318403741736 ) ;
#94345=DIRECTION ( 'NONE',  ( -4.274815082592931898E-19, -0.9999939076577903929, -0.003490651415223739937 ) ) ;
#94346=DIRECTION ( 'NONE',  ( 0.000000000000000000, 1.000000000000000000, 0.000000000000000000 ) ) ;
#94347=PLANE ( 'NONE',  #76228 ) ;
#94348=ORIENTED_EDGE ( 'NONE', *, *, #72342, .F. ) ;
#94349=VERTEX_POINT ( 'NONE', #43461 ) ;
#94350=CARTESIAN_POINT ( 'NONE',  ( -0.4000000000000396572, 2.500000000000000000, 3.637306695894644726 ) ) ;
#94351=ORIENTED_EDGE ( 'NONE', *, *, #43501, .F. ) ;
#94352=DIRECTION ( 'NONE',  ( -0.000000000000000000, 1.000000000000000000, -0.000000000000000000 ) ) ;
#94353=CARTESIAN_POINT ( 'NONE',  ( -5.000000000000024869, 12.50000000000000000, -5.088040615133791356 ) ) ;
#94354=ADVANCED_FACE ( 'NONE', ( #34930 ), #36110, .T. ) ;
#94357=DIRECTION ( 'NONE',  ( 0.000000000000000000, -0.9999939076577903929, 0.003490651415223739937 ) ) ;
#94358=FACE_OUTER_BOUND ( 'NONE', #106991, .T. ) ;
#94359=DIRECTION ( 'NONE',  ( -0.000000000000000000, 1.000000000000000000, -0.000000000000000000 ) ) ;
#94360=DIRECTION ( 'NONE',  ( 0.000000000000000000, 0.000000000000000000, 1.000000000000000000 ) ) ;
#94361=DIRECTION ( 'NONE',  ( 0.000000000000000000, 1.000000000000000000, 0.000000000000000000 ) ) ;
#94363=CARTESIAN_POINT ( 'NONE',  ( 1.049999999999952971, 2.500000000000000000, 6.148780366869520897 ) ) ;
#94364=DIRECTION ( 'NONE',  ( -0.000000000000000000, 1.000000000000000000, -0.000000000000000000 ) ) ;
#94365=VERTEX_POINT ( 'NONE', #73531 ) ;
#94366=ORIENTED_EDGE ( 'NONE', *, *, #119637, .F. ) ;
#94367=ORIENTED_EDGE ( 'NONE', *, *, #2702, .F. ) ;
#94368=CARTESIAN_POINT ( 'NONE',  ( -8.150000000000014566, 12.50000000000000000, -6.906693963081110610 ) ) ;
#94369=ORIENTED_EDGE ( 'NONE', *, *, #31645, .T. ) ;
#94370=CIRCLE ( 'NONE', #21124, 0.1000000000000000056 ) ;
#94371=DIRECTION ( 'NONE',  ( -0.000000000000000000, 1.000000000000000000, -0.000000000000000000 ) ) ;
#94372=AXIS2_PLACEMENT_3D ( 'NONE', #86198, #126142, #94744 ) ;
#94373=CIRCLE ( 'NONE', #123697, 0.09999999999999999167 ) ;
#94374=EDGE_LOOP ( 'NONE', ( #10266, #25736, #68879, #26141 ) ) ;
#94375=ORIENTED_EDGE ( 'NONE', *, *, #45394, .T. ) ;
#94376=EDGE_LOOP ( 'NONE', ( #74906, #19057 ) ) ;
#94377=PLANE ( 'NONE',  #77266 ) ;
#94378=VECTOR ( 'NONE', #110562, 1000.000000000000000 ) ;
#94379=CARTESIAN_POINT ( 'NONE',  ( 5.599999999999931255, 2.500000000000000000, 4.576537180435972019 ) ) ;
#94380=CIRCLE ( 'NONE', #65121, 0.09999999999999982514 ) ;
#94381=LINE ( 'NONE', #15157, #1219 ) ;
#94382=PLANE ( 'NONE',  #85312 ) ;
#94383=AXIS2_PLACEMENT_3D ( 'NONE', #121933, #81381, #82001 ) ;
#94384=CARTESIAN_POINT ( 'NONE',  ( 9.349999999999916156, 2.500000000000000000, 6.841600689897072485 ) ) ;
#94385=ORIENTED_EDGE ( 'NONE', *, *, #39686, .T. ) ;
#94386=CARTESIAN_POINT ( 'NONE',  ( 1.699999999999950218, 2.500000000000000000, 4.430127018922196847 ) ) ;
#94387=ORIENTED_EDGE ( 'NONE', *, *, #80467, .T. ) ;
#94388=VERTEX_POINT ( 'NONE', #74839 ) ;
#94389=ADVANCED_FACE ( 'NONE', ( #122011 ), #52822, .T. ) ;
#94390=EDGE_LOOP ( 'NONE', ( #40218, #39359, #2942, #100012 ) ) ;
#94391=DIRECTION ( 'NONE',  ( 0.000000000000000000, 0.000000000000000000, -1.000000000000000000 ) ) ;
#94392=EDGE_LOOP ( 'NONE', ( #87737, #47371, #119619, #50985 ) ) ;
#94393=ORIENTED_EDGE ( 'NONE', *, *, #69301, .T. ) ;
#94394=ORIENTED_EDGE ( 'NONE', *, *, #20054, .F. ) ;
#94395=DIRECTION ( 'NONE',  ( -0.000000000000000000, 1.000000000000000000, -0.000000000000000000 ) ) ;
#94396=ADVANCED_FACE ( 'NONE', ( #94460 ), #40321, .T. ) ;
#94397=CARTESIAN_POINT ( 'NONE',  ( 14.54999999999989591, 2.500000000000000000, 2.265063509461097357 ) ) ;
#94398=CARTESIAN_POINT ( 'NONE',  ( -14.14999999999998614, 12.50000000000000000, 1.407149913249511997 ) ) ;
#94399=PLANE ( 'NONE',  #121556 ) ;
#94400=DIRECTION ( 'NONE',  ( -0.000000000000000000, 1.000000000000000000, -0.000000000000000000 ) ) ;
#94401=CARTESIAN_POINT ( 'NONE',  ( 4.349999999999941025, 12.50000000000000000, -1.818653347947326138 ) ) ;
#94402=VERTEX_POINT ( 'NONE', #53909 ) ;
#94403=FACE_OUTER_BOUND ( 'NONE', #87252, .T. ) ;
#94404=AXIS2_PLACEMENT_3D ( 'NONE', #32653, #14255, #5081 ) ;
#94405=AXIS2_PLACEMENT_3D ( 'NONE', #25179, #7469, #106327 ) ;
#94406=VERTEX_POINT ( 'NONE', #114113 ) ;
#94407=LINE ( 'NONE', #34881, #81877 ) ;
#94408=ORIENTED_EDGE ( 'NONE', *, *, #122700, .F. ) ;
#94409=DIRECTION ( 'NONE',  ( 0.000000000000000000, 1.000000000000000000, 0.000000000000000000 ) ) ;
#94410=ORIENTED_EDGE ( 'NONE', *, *, #109405, .F. ) ;
#94411=EDGE_LOOP ( 'NONE', ( #99538, #3557, #121016, #32244 ) ) ;
#94412=CONICAL_SURFACE ( 'NONE', #98516, 0.1000000000000002554, 0.003490658503988666988 ) ;
#94413=DIRECTION ( 'NONE',  ( -4.274815082592931898E-19, -0.9999939076577903929, -0.003490651415223739937 ) ) ;
#94414=DIRECTION ( 'NONE',  ( 0.000000000000000000, 1.000000000000000000, 0.000000000000000000 ) ) ;
#94415=VECTOR ( 'NONE', #16940, 1000.000000000000000 ) ;
#94416=CONICAL_SURFACE ( 'NONE', #102726, 0.09999999999999999167, 0.003490658503988666988 ) ;
#94417=CARTESIAN_POINT ( 'NONE',  ( -7.500000000000016875, 2.500000000000000000, -3.637306695894650055 ) ) ;
#94418=EDGE_LOOP ( 'NONE', ( #23996, #99022, #107441, #44004 ) ) ;
#94419=LINE ( 'NONE', #82204, #65878 ) ;
#94420=ORIENTED_EDGE ( 'NONE', *, *, #116844, .F. ) ;
#94421=CARTESIAN_POINT ( 'NONE',  ( -9.150000000000009237, 2.500000000000000000, -2.265063509461101798 ) ) ;
#94422=CARTESIAN_POINT ( 'NONE',  ( -1.650000000000035660, 2.500000000000000000, 7.288010851410849256 ) ) ;
#94423=PLANE ( 'NONE',  #73194 ) ;
#94424=CARTESIAN_POINT ( 'NONE',  ( -9.150000000000011013, 2.500000000000000000, -5.802370205355744659 ) ) ;
#94425=VECTOR ( 'NONE', #58585, 1000.000000000000000 ) ;
#94427=CARTESIAN_POINT ( 'NONE',  ( 6.699999999999928235, 12.50000000000000000, -0.06509327318403970719 ) ) ;
#94428=EDGE_CURVE ( 'NONE', #43830, #72875, #29845, .T. ) ;
#94429=ORIENTED_EDGE ( 'NONE', *, *, #106786, .F. ) ;
#94430=CIRCLE ( 'NONE', #109187, 0.06509327318403745899 ) ;
#94431=VECTOR ( 'NONE', #68438, 1000.000000000000000 ) ;
#94432=AXIS2_PLACEMENT_3D ( 'NONE', #77567, #118149, #97860 ) ;
#94433=ORIENTED_EDGE ( 'NONE', *, *, #53577, .T. ) ;
#94434=FACE_OUTER_BOUND ( 'NONE', #22160, .T. ) ;
#94435=DIRECTION ( 'NONE',  ( -0.000000000000000000, 1.000000000000000000, -0.000000000000000000 ) ) ;
#94436=ADVANCED_FACE ( 'NONE', ( #123290 ), #74195, .T. ) ;
#94437=EDGE_CURVE ( 'NONE', #39788, #64883, #124585, .T. ) ;
#94439=CARTESIAN_POINT ( 'NONE',  ( 1.249999999999953815, 2.500000000000000000, -2.957883832488653830 ) ) ;
#94440=DIRECTION ( 'NONE',  ( 0.000000000000000000, 0.000000000000000000, 1.000000000000000000 ) ) ;
#94441=CARTESIAN_POINT ( 'NONE',  ( 3.149999999999946176, 2.500000000000000000, -1.818653347947325916 ) ) ;
#94442=EDGE_CURVE ( 'NONE', #34687, #118817, #25720, .T. ) ;
#94443=DIRECTION ( 'NONE',  ( 0.000000000000000000, -0.9999939076577903929, 0.003490651415223739937 ) ) ;
#94444=ORIENTED_EDGE ( 'NONE', *, *, #68202, .F. ) ;
#94445=CARTESIAN_POINT ( 'NONE',  ( -10.65000000000000391, 2.500000000000000000, -6.941600689897075682 ) ) ;
#94446=B_SPLINE_CURVE_WITH_KNOTS ( 'NONE', 3,
 ( #107873, #86943, #96749, #127523, #106581, #38517, #16875, #48313 ),
 .UNSPECIFIED., .F., .F.,
 ( 4, 2, 2, 4 ),
 ( 0.000000000000000000, 0.001904977314310103524, 0.002857465971465155286, 0.003809954628620207048 ),
 .UNSPECIFIED. ) ;
#94447=DIRECTION ( 'NONE',  ( -0.000000000000000000, 1.000000000000000000, -0.000000000000000000 ) ) ;
#94448=DIRECTION ( 'NONE',  ( -0.000000000000000000, -1.000000000000000000, -0.000000000000000000 ) ) ;
#94449=ADVANCED_FACE ( 'NONE', ( #32370 ), #98880, .T. ) ;
#94450=EDGE_LOOP ( 'NONE', ( #123706, #65491 ) ) ;
#94451=EDGE_CURVE ( 'NONE', #119417, #72819, #48821, .T. ) ;
#94453=ORIENTED_EDGE ( 'NONE', *, *, #126272, .T. ) ;
#94454=CARTESIAN_POINT ( 'NONE',  ( 2.099999999999949463, 2.500000000000000000, 0.6928203230275494784 ) ) ;
#94455=AXIS2_PLACEMENT_3D ( 'NONE', #90946, #1273, #123610 ) ;
#94456=AXIS2_PLACEMENT_3D ( 'NONE', #110991, #101843, #11524 ) ;
#94457=VECTOR ( 'NONE', #74137, 1000.000000000000000 ) ;
#94458=EDGE_LOOP ( 'NONE', ( #34795, #32884 ) ) ;
#94459=DIRECTION ( 'NONE',  ( 0.000000000000000000, 0.000000000000000000, 1.000000000000000000 ) ) ;
#94460=FACE_OUTER_BOUND ( 'NONE', #77954, .T. ) ;
#94461=DIRECTION ( 'NONE',  ( -0.000000000000000000, -1.000000000000000000, -0.000000000000000000 ) ) ;
#94462=ORIENTED_EDGE ( 'NONE', *, *, #116381, .T. ) ;
#94465=AXIS2_PLACEMENT_3D ( 'NONE', #26940, #23220, #63153 ) ;
#94466=FACE_OUTER_BOUND ( 'NONE', #14250, .T. ) ;
#94467=VECTOR ( 'NONE', #122712, 1000.000000000000000 ) ;
#94468=CIRCLE ( 'NONE', #102782, 0.06509327318403745899 ) ;
#94469=ORIENTED_EDGE ( 'NONE', *, *, #37170, .T. ) ;
#94470=CIRCLE ( 'NONE', #19156, 0.1000000000000002554 ) ;
#94471=DIRECTION ( 'NONE',  ( 0.000000000000000000, 0.000000000000000000, -1.000000000000000000 ) ) ;
#94472=ORIENTED_EDGE ( 'NONE', *, *, #98179, .T. ) ;
#94473=ORIENTED_EDGE ( 'NONE', *, *, #68314, .T. ) ;
#94474=CARTESIAN_POINT ( 'NONE',  ( 11.04999999999990656, 12.50000000000000000, 2.511473670974873507 ) ) ;
#94475=CARTESIAN_POINT ( 'NONE',  ( -0.6000000000000323963, 2.500000000000000000, 0.2464101615137759549 ) ) ;
#94476=ORIENTED_EDGE ( 'NONE', *, *, #12863, .T. ) ;
#94477=DIRECTION ( 'NONE',  ( -4.274815082592931898E-19, -0.9999939076577903929, -0.003490651415223739937 ) ) ;
#94478=DIRECTION ( 'NONE',  ( -4.274815082592931898E-19, -0.9999939076577903929, -0.003490651415223739937 ) ) ;
#94479=ORIENTED_EDGE ( 'NONE', *, *, #91388, .T. ) ;
#94480=EDGE_CURVE ( 'NONE', #59346, #38624, #91900, .T. ) ;
#94481=CARTESIAN_POINT ( 'NONE',  ( 9.999999999999916511, 2.500000000000000000, -0.7928203230275542301 ) ) ;
#94482=CARTESIAN_POINT ( 'NONE',  ( 8.749999999999918288, 2.500000000000000000, 7.188010851410848723 ) ) ;
#94483=DIRECTION ( 'NONE',  ( -4.274815082592931898E-19, -0.9999939076577903929, -0.003490651415223739937 ) ) ;
#94484=ADVANCED_FACE ( 'NONE', ( #104298 ), #82072, .T. ) ;
#94485=CARTESIAN_POINT ( 'NONE',  ( 17.49149641758750562, -2.499999999999849010, -4.292093396893348789 ) ) ;
#94486=CARTESIAN_POINT ( 'NONE',  ( -14.14999999999998614, 2.500000000000000000, 1.572243186433549544 ) ) ;
#94487=ADVANCED_FACE ( 'NONE', ( #63081 ), #94772, .T. ) ;
#94488=DIRECTION ( 'NONE',  ( 0.000000000000000000, 0.000000000000000000, 1.000000000000000000 ) ) ;
#94489=DIRECTION ( 'NONE',  ( 0.000000000000000000, 0.000000000000000000, 1.000000000000000000 ) ) ;
#94490=EDGE_CURVE ( 'NONE', #1350, #110433, #4780, .T. ) ;
#94491=ADVANCED_FACE ( 'NONE', ( #32996 ), #113555, .T. ) ;
#94492=AXIS2_PLACEMENT_3D ( 'NONE', #69153, #79631, #109062 ) ;
#94493=VECTOR ( 'NONE', #83940, 1000.000000000000000 ) ;
#94494=EDGE_LOOP ( 'NONE', ( #112276, #94174 ) ) ;
#94495=VERTEX_POINT ( 'NONE', #23152 ) ;
#94496=EDGE_CURVE ( 'NONE', #103868, #17323, #46661, .T. ) ;
#94497=ORIENTED_EDGE ( 'NONE', *, *, #69141, .T. ) ;
#94498=EDGE_LOOP ( 'NONE', ( #25235, #100240 ) ) ;
#94499=LINE ( 'NONE', #114785, #62061 ) ;
#94500=CARTESIAN_POINT ( 'NONE',  ( -0.4500000000000397571, 2.500000000000000000, -6.495190528383302464 ) ) ;
#94501=CARTESIAN_POINT ( 'NONE',  ( -13.94999999999998863, 2.500000000000000000, 2.511473670974877503 ) ) ;
#94502=ORIENTED_EDGE ( 'NONE', *, *, #60767, .T. ) ;
#94503=FACE_BOUND ( 'NONE', #87012, .T. ) ;
#94504=AXIS2_PLACEMENT_3D ( 'NONE', #109770, #79657, #59404 ) ;
#94505=DIRECTION ( 'NONE',  ( 0.000000000000000000, 0.000000000000000000, 1.000000000000000000 ) ) ;
#94506=CARTESIAN_POINT ( 'NONE',  ( 10.44999999999991402, 2.500000000000000000, -2.165063509461101710 ) ) ;
#94507=AXIS2_PLACEMENT_3D ( 'NONE', #45481, #23900, #63821 ) ;
#94508=EDGE_CURVE ( 'NONE', #34729, #45548, #17387, .T. ) ;
#94509=CIRCLE ( 'NONE', #6651, 0.1000000000000002554 ) ;
#94510=DIRECTION ( 'NONE',  ( 0.000000000000000000, 0.000000000000000000, -1.000000000000000000 ) ) ;
#94511=EDGE_CURVE ( 'NONE', #53510, #120782, #35566, .T. ) ;
#94512=VECTOR ( 'NONE', #73661, 1000.000000000000000 ) ;
#94513=LINE ( 'NONE', #76822, #15740 ) ;
#94514=DIRECTION ( 'NONE',  ( 0.000000000000000000, 1.000000000000000000, 0.000000000000000000 ) ) ;
#94515=PLANE ( 'NONE',  #9930 ) ;
#94516=CARTESIAN_POINT ( 'NONE',  ( -11.64999999999999680, 2.500000000000000000, -6.495190528383298911 ) ) ;
#94517=CARTESIAN_POINT ( 'NONE',  ( 1.649999999999950617, 2.500000000000000000, -2.165063509461101710 ) ) ;
#94518=CARTESIAN_POINT ( 'NONE',  ( 6.249999999999968914, 12.50000000000000000, -6.495190528383302464 ) ) ;
#94519=AXIS2_PLACEMENT_3D ( 'NONE', #104136, #120076, #50066 ) ;
#94520=CARTESIAN_POINT ( 'NONE',  ( -4.350000000000023626, 2.500000000000000000, -1.818653347947325916 ) ) ;
#94521=AXIS2_PLACEMENT_3D ( 'NONE', #24307, #35428, #43956 ) ;
#94522=EDGE_LOOP ( 'NONE', ( #110179, #121967 ) ) ;
#94523=ORIENTED_EDGE ( 'NONE', *, *, #3963, .F. ) ;
#94524=EDGE_LOOP ( 'NONE', ( #974, #95033 ) ) ;
#94525=AXIS2_PLACEMENT_3D ( 'NONE', #66315, #97072, #85942 ) ;
#94526=VERTEX_POINT ( 'NONE', #57782 ) ;
#94527=AXIS2_PLACEMENT_3D ( 'NONE', #96974, #129046, #7294 ) ;
#94528=CIRCLE ( 'NONE', #107035, 0.09999999999999999167 ) ;
#94529=DIRECTION ( 'NONE',  ( 0.000000000000000000, 1.000000000000000000, 0.000000000000000000 ) ) ;
#94530=ORIENTED_EDGE ( 'NONE', *, *, #12811, .F. ) ;
#94531=FACE_OUTER_BOUND ( 'NONE', #8680, .T. ) ;
#94532=ORIENTED_EDGE ( 'NONE', *, *, #84990, .T. ) ;
#94533=EDGE_LOOP ( 'NONE', ( #199, #117878 ) ) ;
#94534=CIRCLE ( 'NONE', #63147, 0.06509327318403745899 ) ;
#94535=AXIS2_PLACEMENT_3D ( 'NONE', #31420, #40617, #32723 ) ;
#94536=CARTESIAN_POINT ( 'NONE',  ( 7.314170287631764467, -1.500000000000000222, 9.688393442221800100 ) ) ;
#94537=FACE_OUTER_BOUND ( 'NONE', #46676, .T. ) ;
#94538=DIRECTION ( 'NONE',  ( 0.000000000000000000, 0.000000000000000000, 1.000000000000000000 ) ) ;
#94539=CARTESIAN_POINT ( 'NONE',  ( 6.649999999999929301, 12.50000000000000000, -2.165063509461101710 ) ) ;
#94540=VERTEX_POINT ( 'NONE', #36212 ) ;
#94541=VERTEX_POINT ( 'NONE', #27029 ) ;
#94542=ORIENTED_EDGE ( 'NONE', *, *, #20456, .T. ) ;
#94543=DIRECTION ( 'NONE',  ( -4.274815082592931898E-19, -0.9999939076577903929, -0.003490651415223739937 ) ) ;
#94544=ORIENTED_EDGE ( 'NONE', *, *, #37558, .T. ) ;
#94545=DIRECTION ( 'NONE',  ( 0.000000000000000000, 1.000000000000000000, 0.000000000000000000 ) ) ;
#94546=ORIENTED_EDGE ( 'NONE', *, *, #72415, .T. ) ;
#94547=ORIENTED_EDGE ( 'NONE', *, *, #46757, .F. ) ;
#94548=DIRECTION ( 'NONE',  ( 0.000000000000000000, 0.000000000000000000, 1.000000000000000000 ) ) ;
#94549=EDGE_CURVE ( 'NONE', #112302, #21997, #116683, .T. ) ;
#94550=CARTESIAN_POINT ( 'NONE',  ( -15.59999999999998010, 2.500000000000000000, -0.4464101615137759382 ) ) ;
#94551=CARTESIAN_POINT ( 'NONE',  ( -1.850000000000033396, 2.500000000000000000, -1.918653347947325782 ) ) ;
#94552=AXIS2_PLACEMENT_3D ( 'NONE', #48947, #79055, #20119 ) ;
#94553=DIRECTION ( 'NONE',  ( 0.000000000000000000, 1.000000000000000000, 0.000000000000000000 ) ) ;
#94554=VECTOR ( 'NONE', #129020, 1000.000000000000000 ) ;
#94555=CIRCLE ( 'NONE', #10907, 0.06509327318403745899 ) ;
#94556=PLANE ( 'NONE',  #8492 ) ;
#94557=ORIENTED_EDGE ( 'NONE', *, *, #31062, .T. ) ;
#94558=DIRECTION ( 'NONE',  ( 0.000000000000000000, 0.000000000000000000, 1.000000000000000000 ) ) ;
#94559=CIRCLE ( 'NONE', #6799, 0.1000000000000002554 ) ;
#94560=EDGE_LOOP ( 'NONE', ( #629, #74951, #102689, #79713 ) ) ;
#94561=DIRECTION ( 'NONE',  ( -0.000000000000000000, -1.000000000000000000, -0.000000000000000000 ) ) ;
#94562=CONICAL_SURFACE ( 'NONE', #123794, 0.1000000000000002554, 0.003490658503988666988 ) ;
#94563=VERTEX_POINT ( 'NONE', #87218 ) ;
#94564=CARTESIAN_POINT ( 'NONE',  ( 13.09999999999990195, 12.50000000000000000, -4.611443907251940644 ) ) ;
#94565=DIRECTION ( 'NONE',  ( 0.000000000000000000, 0.000000000000000000, 1.000000000000000000 ) ) ;
#94566=AXIS2_PLACEMENT_3D ( 'NONE', #34999, #4202, #74905 ) ;
#94567=CARTESIAN_POINT ( 'NONE',  ( 10.59999999999991260, 2.500000000000000000, -0.3464101615137783474 ) ) ;
#94568=DIRECTION ( 'NONE',  ( -0.000000000000000000, -1.000000000000000000, -0.000000000000000000 ) ) ;
#94569=EDGE_LOOP ( 'NONE', ( #48916, #9306 ) ) ;
#94570=CIRCLE ( 'NONE', #102882, 0.06509327318403745899 ) ;
#94571=SURFACE_SIDE_STYLE ('',( #45499 ) ) ;
#94572=CARTESIAN_POINT ( 'NONE',  ( 9.399999999999915090, 2.500000000000000000, -3.983716857408426293 ) ) ;
#94573=EDGE_LOOP ( 'NONE', ( #95445, #95798, #119537, #97830 ) ) ;
#94574=ORIENTED_EDGE ( 'NONE', *, *, #54583, .T. ) ;
#94575=ORIENTED_EDGE ( 'NONE', *, *, #112280, .F. ) ;
#94576=CARTESIAN_POINT ( 'NONE',  ( -13.34999999999999076, 2.500000000000000000, -2.265063509461099578 ) ) ;
#94577=CARTESIAN_POINT ( 'NONE',  ( 8.149999999999920419, 12.50000000000000000, -1.818653347947325916 ) ) ;
#94579=DIRECTION ( 'NONE',  ( -0.000000000000000000, 1.000000000000000000, -0.000000000000000000 ) ) ;
#94580=VECTOR ( 'NONE', #107821, 1000.000000000000000 ) ;
#94581=CARTESIAN_POINT ( 'NONE',  ( 8.949999999999917577, 2.500000000000000000, 6.148780366869520009 ) ) ;
#94582=LINE ( 'NONE', #4911, #38246 ) ;
#94583=VERTEX_POINT ( 'NONE', #95765 ) ;
#94584=DIRECTION ( 'NONE',  ( 0.000000000000000000, 0.000000000000000000, 1.000000000000000000 ) ) ;
#94585=EDGE_CURVE ( 'NONE', #56480, #59007, #109347, .T. ) ;
#94586=ORIENTED_EDGE ( 'NONE', *, *, #33531, .F. ) ;
#94587=ADVANCED_FACE ( 'NONE', ( #85293 ), #101039, .T. ) ;
#94588=CARTESIAN_POINT ( 'NONE',  ( -0.6500000000000398792, 2.500000000000000000, -2.411473670974877859 ) ) ;
#94590=LINE ( 'NONE', #54042, #77287 ) ;
#94591=VECTOR ( 'NONE', #27820, 1000.000000000000000 ) ;
#94592=ADVANCED_FACE ( 'NONE', ( #106852 ), #92628, .T. ) ;
#94593=CIRCLE ( 'NONE', #50690, 0.06509327318403745899 ) ;
#94594=EDGE_LOOP ( 'NONE', ( #33582, #45340 ) ) ;
#94595=CONICAL_SURFACE ( 'NONE', #117564, 0.09999999999999982514, 0.003490658503988666988 ) ;
#94596=CONICAL_SURFACE ( 'NONE', #15167, 0.1000000000000002554, 0.003490658503988666988 ) ;
#94598=DIRECTION ( 'NONE',  ( 0.000000000000000000, 0.000000000000000000, 1.000000000000000000 ) ) ;
#94599=ADVANCED_FACE ( 'NONE', ( #47313 ), #26391, .T. ) ;
#94600=ADVANCED_FACE ( 'NONE', ( #16534 ), #44600, .T. ) ;
#94601=EDGE_CURVE ( 'NONE', #21869, #110514, #67566, .T. ) ;
#94602=ADVANCED_FACE ( 'NONE', ( #46666 ), #23669, .T. ) ;
#94603=ORIENTED_EDGE ( 'NONE', *, *, #86303, .T. ) ;
#94604=DIRECTION ( 'NONE',  ( 0.000000000000000000, -0.000000000000000000, 1.000000000000000000 ) ) ;
#94605=AXIS2_PLACEMENT_3D ( 'NONE', #70040, #100149, #40608 ) ;
#94606=ORIENTED_EDGE ( 'NONE', *, *, #110627, .F. ) ;
#94607=AXIS2_PLACEMENT_3D ( 'NONE', #58829, #120330, #20839 ) ;
#94608=CIRCLE ( 'NONE', #52758, 0.06509327318403745899 ) ;
#94609=VERTEX_POINT ( 'NONE', #97054 ) ;
#94611=DIRECTION ( 'NONE',  ( 0.000000000000000000, 1.000000000000000000, 0.000000000000000000 ) ) ;
#94612=EDGE_CURVE ( 'NONE', #46131, #129259, #678, .T. ) ;
#94613=AXIS2_PLACEMENT_3D ( 'NONE', #90801, #80349, #67934 ) ;
#94614=ORIENTED_EDGE ( 'NONE', *, *, #95815, .F. ) ;
#94615=DIRECTION ( 'NONE',  ( 0.000000000000000000, 0.000000000000000000, 1.000000000000000000 ) ) ;
#94617=DIRECTION ( 'NONE',  ( 0.000000000000000000, -0.9999939076577903929, 0.003490651415223739937 ) ) ;
#94618=ORIENTED_EDGE ( 'NONE', *, *, #116176, .F. ) ;
#94619=FACE_BOUND ( 'NONE', #19732, .T. ) ;
#94620=AXIS2_PLACEMENT_3D ( 'NONE', #42373, #82303, #29983 ) ;
#94621=CARTESIAN_POINT ( 'NONE',  ( 9.799999999999913669, 2.500000000000000000, 4.676537180435972552 ) ) ;
#94622=DIRECTION ( 'NONE',  ( -4.274815082592931898E-19, -0.9999939076577903929, -0.003490651415223739937 ) ) ;
#94623=ORIENTED_EDGE ( 'NONE', *, *, #50906, .T. ) ;
#94624=DIRECTION ( 'NONE',  ( 0.000000000000000000, 1.000000000000000000, 0.000000000000000000 ) ) ;
#94625=CARTESIAN_POINT ( 'NONE',  ( -7.300000000000018474, 12.50000000000000000, -4.048810130592463530 ) ) ;
#94626=ORIENTED_EDGE ( 'NONE', *, *, #111878, .T. ) ;
#94627=EDGE_LOOP ( 'NONE', ( #40552, #88873 ) ) ;
#94628=ORIENTED_EDGE ( 'NONE', *, *, #122795, .F. ) ;
#94629=DIRECTION ( 'NONE',  ( -0.000000000000000000, -1.000000000000000000, -0.000000000000000000 ) ) ;
#94630=CARTESIAN_POINT ( 'NONE',  ( -4.400000000000028777, 2.500000000000000000, -4.676537180435978769 ) ) ;
#94631=CARTESIAN_POINT ( 'NONE',  ( 7.099999999999927702, 2.500000000000000000, 5.022947341949748790 ) ) ;
#94632=AXIS2_PLACEMENT_3D ( 'NONE', #3956, #43903, #34077 ) ;
#94633=FACE_BOUND ( 'NONE', #30464, .T. ) ;
#94634=ORIENTED_EDGE ( 'NONE', *, *, #12843, .T. ) ;
#94636=CARTESIAN_POINT ( 'NONE',  ( 10.59999999999991260, 2.500000000000000000, -0.3464101615137783474 ) ) ;
#94637=DIRECTION ( 'NONE',  ( 0.000000000000000000, 0.000000000000000000, -1.000000000000000000 ) ) ;
#94638=FACE_OUTER_BOUND ( 'NONE', #74420, .T. ) ;
#94639=AXIS2_PLACEMENT_3D ( 'NONE', #88027, #38327, #65171 ) ;
#94640=CARTESIAN_POINT ( 'NONE',  ( -5.400000000000019895, 2.500000000000000000, 3.737306695894644371 ) ) ;
#94641=VECTOR ( 'NONE', #3936, 1000.000000000000000 ) ;
#94642=CARTESIAN_POINT ( 'NONE',  ( -1.050000000000038236, 2.500000000000000000, -6.248780366869526759 ) ) ;
#94643=ADVANCED_FACE ( 'NONE', ( #105594 ), #80114, .T. ) ;
#94644=FACE_OUTER_BOUND ( 'NONE', #91387, .T. ) ;
#94645=EDGE_CURVE ( 'NONE', #114219, #67325, #96820, .T. ) ;
#94646=CONICAL_SURFACE ( 'NONE', #31985, 0.1000000000000002554, 0.003490658503988666988 ) ;
#94647=CARTESIAN_POINT ( 'NONE',  ( -14.99999999999994671, 12.50000000000000000, 0.000000000000000000 ) ) ;
#94648=EDGE_CURVE ( 'NONE', #84209, #20024, #21620, .T. ) ;
#94649=AXIS2_PLACEMENT_3D ( 'NONE', #46797, #66417, #125346 ) ;
#94650=VERTEX_POINT ( 'NONE', #117970 ) ;
#94651=EDGE_LOOP ( 'NONE', ( #98159, #90896 ) ) ;
#94652=ORIENTED_EDGE ( 'NONE', *, *, #48590, .T. ) ;
#94653=ORIENTED_EDGE ( 'NONE', *, *, #32658, .F. ) ;
#94654=AXIS2_PLACEMENT_3D ( 'NONE', #81979, #32270, #29665 ) ;
#94655=VERTEX_POINT ( 'NONE', #5436 ) ;
#94656=DIRECTION ( 'NONE',  ( 0.000000000000000000, -0.000000000000000000, 1.000000000000000000 ) ) ;
#94657=VECTOR ( 'NONE', #33248, 1000.000000000000000 ) ;
#94658=LINE ( 'NONE', #35126, #113495 ) ;
#94659=ORIENTED_EDGE ( 'NONE', *, *, #68573, .F. ) ;
#94660=EDGE_CURVE ( 'NONE', #31405, #59442, #15332, .T. ) ;
#94661=FACE_BOUND ( 'NONE', #104609, .T. ) ;
#94662=VECTOR ( 'NONE', #54807, 1000.000000000000000 ) ;
#94663=LINE ( 'NONE', #123476, #31076 ) ;
#94664=EDGE_CURVE ( 'NONE', #43749, #104669, #32099, .T. ) ;
#94665=EDGE_CURVE ( 'NONE', #103959, #7038, #48729, .T. ) ;
#94666=EDGE_CURVE ( 'NONE', #109430, #96170, #86353, .T. ) ;
#94667=DIRECTION ( 'NONE',  ( 0.000000000000000000, 0.000000000000000000, 1.000000000000000000 ) ) ;
#94668=VERTEX_POINT ( 'NONE', #119258 ) ;
#94669=DIRECTION ( 'NONE',  ( 0.000000000000000000, 0.000000000000000000, -1.000000000000000000 ) ) ;
#94671=CARTESIAN_POINT ( 'NONE',  ( 12.49999999999990230, 2.500000000000000000, -0.7928203230275542301 ) ) ;
#94672=ORIENTED_EDGE ( 'NONE', *, *, #46165, .F. ) ;
#94673=CARTESIAN_POINT ( 'NONE',  ( -6.900000000000019007, 2.500000000000000000, 0.3464101615137735735 ) ) ;
#94674=EDGE_CURVE ( 'NONE', #69453, #94894, #8991, .T. ) ;
#94675=AXIS2_PLACEMENT_3D ( 'NONE', #120075, #9472, #1573 ) ;
#94676=VERTEX_POINT ( 'NONE', #110725 ) ;
#94677=VERTEX_POINT ( 'NONE', #773 ) ;
#94678=VERTEX_POINT ( 'NONE', #99636 ) ;
#94679=DIRECTION ( 'NONE',  ( -0.000000000000000000, 1.000000000000000000, -0.000000000000000000 ) ) ;
#94680=CARTESIAN_POINT ( 'NONE',  ( -7.900000000000014566, 2.500000000000000000, -4.330127018922201643 ) ) ;
#94682=ORIENTED_EDGE ( 'NONE', *, *, #66978, .F. ) ;
#94683=CARTESIAN_POINT ( 'NONE',  ( 2.500000000000002220, 2.499999999999998668, -9.999999999999998224 ) ) ;
#94684=CIRCLE ( 'NONE', #38268, 0.06509327318403745899 ) ;
#94685=AXIS2_PLACEMENT_3D ( 'NONE', #37381, #77930, #98856 ) ;
#94686=FACE_OUTER_BOUND ( 'NONE', #12278, .T. ) ;
#94687=DIRECTION ( 'NONE',  ( 0.000000000000000000, 0.000000000000000000, 1.000000000000000000 ) ) ;
#94689=CARTESIAN_POINT ( 'NONE',  ( 3.149999999999946176, 12.50000000000000000, -1.883746621131363375 ) ) ;
#94690=DIRECTION ( 'NONE',  ( -4.274815082592931898E-19, -0.9999939076577903929, -0.003490651415223739937 ) ) ;
#94691=ADVANCED_FACE ( 'NONE', ( #21056 ), #29596, .T. ) ;
#94692=ORIENTED_EDGE ( 'NONE', *, *, #95051, .F. ) ;
#94693=FACE_OUTER_BOUND ( 'NONE', #24659, .T. ) ;
#94695=AXIS2_PLACEMENT_3D ( 'NONE', #66823, #28209, #26919 ) ;
#94696=ORIENTED_EDGE ( 'NONE', *, *, #51225, .T. ) ;
#94697=CONICAL_SURFACE ( 'NONE', #90486, 0.09999999999999999167, 0.003490658503988666988 ) ;
#94698=ORIENTED_EDGE ( 'NONE', *, *, #113030, .T. ) ;
#94699=CARTESIAN_POINT ( 'NONE',  ( 4.999999999999938716, 2.500000000000000000, -5.022947341949754119 ) ) ;
#94700=DIRECTION ( 'NONE',  ( 0.000000000000000000, 1.000000000000000000, 0.000000000000000000 ) ) ;
#94701=CARTESIAN_POINT ( 'NONE',  ( 13.54999999999989946, 2.500000000000000000, 2.511473670974873507 ) ) ;
#94702=CARTESIAN_POINT ( 'NONE',  ( -8.350000000000012079, 2.500000000000000000, -1.572243186433550211 ) ) ;
#94703=DIRECTION ( 'NONE',  ( 0.000000000000000000, -0.000000000000000000, 1.000000000000000000 ) ) ;
#94704=AXIS2_PLACEMENT_3D ( 'NONE', #24784, #64696, #25398 ) ;
#94705=ORIENTED_EDGE ( 'NONE', *, *, #39169, .F. ) ;
#94706=ORIENTED_EDGE ( 'NONE', *, *, #46463, .T. ) ;
#94707=DIRECTION ( 'NONE',  ( 0.000000000000000000, -0.000000000000000000, 1.000000000000000000 ) ) ;
#94708=EDGE_CURVE ( 'NONE', #12428, #76477, #90429, .T. ) ;
#94709=DIRECTION ( 'NONE',  ( 0.000000000000000000, -0.9999939076577903929, 0.003490651415223739937 ) ) ;
#94710=AXIS2_PLACEMENT_3D ( 'NONE', #72528, #112451, #22149 ) ;
#94711=VECTOR ( 'NONE', #92644, 1000.000000000000000 ) ;
#94712=LINE ( 'NONE', #25313, #112973 ) ;
#94713=ORIENTED_EDGE ( 'NONE', *, *, #119742, .F. ) ;
#94714=ORIENTED_EDGE ( 'NONE', *, *, #84997, .T. ) ;
#94715=CARTESIAN_POINT ( 'NONE',  ( 5.649999999999934630, 2.500000000000000000, -1.718653347947325827 ) ) ;
#94716=AXIS2_PLACEMENT_3D ( 'NONE', #88870, #90136, #39792 ) ;
#94717=ORIENTED_EDGE ( 'NONE', *, *, #105764, .T. ) ;
#94718=CARTESIAN_POINT ( 'NONE',  ( -7.500000000000013323, 2.500000000000000000, 4.922947341949748257 ) ) ;
#94719=DIRECTION ( 'NONE',  ( 0.000000000000000000, 1.000000000000000000, 0.000000000000000000 ) ) ;
#94720=ORIENTED_EDGE ( 'NONE', *, *, #106725, .T. ) ;
#94721=CIRCLE ( 'NONE', #82210, 0.06509327318403745899 ) ;
#94722=CARTESIAN_POINT ( 'NONE',  ( 0.1999999999999576006, 12.50000000000000000, -4.676537180435978769 ) ) ;
#94723=CARTESIAN_POINT ( 'NONE',  ( 5.399999999999936406, 12.50000000000000000, -5.022947341949754119 ) ) ;
#94724=CARTESIAN_POINT ( 'NONE',  ( 3.749999999999940492, 12.50000000000000000, 2.857883832488649301 ) ) ;
#94725=EDGE_CURVE ( 'NONE', #97446, #54303, #19788, .T. ) ;
#94726=CARTESIAN_POINT ( 'NONE',  ( -6.249999999999984901, 2.500000000000000000, -6.395190528383301931 ) ) ;
#94727=EDGE_LOOP ( 'NONE', ( #61700, #6119 ) ) ;
#94728=LINE ( 'NONE', #55458, #121891 ) ;
#94729=DIRECTION ( 'NONE',  ( -0.000000000000000000, 1.000000000000000000, -0.000000000000000000 ) ) ;
#94730=ORIENTED_EDGE ( 'NONE', *, *, #38153, .T. ) ;
#94731=ORIENTED_EDGE ( 'NONE', *, *, #100387, .T. ) ;
#94732=CIRCLE ( 'NONE', #52973, 0.09999999999999982514 ) ;
#94733=AXIS2_PLACEMENT_3D ( 'NONE', #69309, #11691, #9763 ) ;
#94735=DIRECTION ( 'NONE',  ( 0.000000000000000000, -0.000000000000000000, 1.000000000000000000 ) ) ;
#94736=DIRECTION ( 'NONE',  ( 0.000000000000000000, 1.000000000000000000, 0.000000000000000000 ) ) ;
#94737=DIRECTION ( 'NONE',  ( 0.000000000000000000, 0.000000000000000000, 1.000000000000000000 ) ) ;
#94738=CARTESIAN_POINT ( 'NONE',  ( -11.05000000000000249, 2.500000000000000000, -1.918653347947322230 ) ) ;
#94739=VECTOR ( 'NONE', #107671, 1000.000000000000000 ) ;
#94740=DIRECTION ( 'NONE',  ( 0.000000000000000000, 0.000000000000000000, -1.000000000000000000 ) ) ;
#94741=VECTOR ( 'NONE', #57646, 1000.000000000000000 ) ;
#94742=DIRECTION ( 'NONE',  ( 0.000000000000000000, -0.9999939076577903929, 0.003490651415223739937 ) ) ;
#94743=DIRECTION ( 'NONE',  ( 0.000000000000000000, 0.000000000000000000, 1.000000000000000000 ) ) ;
#94744=DIRECTION ( 'NONE',  ( 0.000000000000000000, 0.000000000000000000, 1.000000000000000000 ) ) ;
#94745=CIRCLE ( 'NONE', #40386, 0.1000000000000002554 ) ;
#94746=AXIS2_PLACEMENT_3D ( 'NONE', #115493, #65757, #114229 ) ;
#94747=CARTESIAN_POINT ( 'NONE',  ( -5.850000000000019185, 12.50000000000000000, 6.495190528383297135 ) ) ;
#94748=EDGE_LOOP ( 'NONE', ( #64907, #99265, #91870, #109563 ) ) ;
#94749=CONICAL_SURFACE ( 'NONE', #126147, 0.1000000000000002554, 0.003490658503988666988 ) ;
#94750=VERTEX_POINT ( 'NONE', #88506 ) ;
#94751=CIRCLE ( 'NONE', #11214, 0.1000000000000002554 ) ;
#94752=CONICAL_SURFACE ( 'NONE', #84289, 0.1000000000000002554, 0.003490658503988666988 ) ;
#94753=ADVANCED_FACE ( 'NONE', ( #100901 ), #69511, .T. ) ;
#94754=ORIENTED_EDGE ( 'NONE', *, *, #49552, .T. ) ;
#94755=VECTOR ( 'NONE', #1806, 1000.000000000000000 ) ;
#94756=AXIS2_PLACEMENT_3D ( 'NONE', #28909, #26330, #96991 ) ;
#94757=ORIENTED_EDGE ( 'NONE', *, *, #44111, .F. ) ;
#94758=DIRECTION ( 'NONE',  ( -0.000000000000000000, -1.000000000000000000, -0.000000000000000000 ) ) ;
#94759=DIRECTION ( 'NONE',  ( 0.000000000000000000, 0.000000000000000000, 1.000000000000000000 ) ) ;
#94760=CARTESIAN_POINT ( 'NONE',  ( 11.84999999999990372, 12.50000000000000000, -6.841600689897078702 ) ) ;
#94761=AXIS2_PLACEMENT_3D ( 'NONE', #67520, #47922, #127756 ) ;
#94762=EDGE_CURVE ( 'NONE', #88981, #22544, #98324, .T. ) ;
#94763=ORIENTED_EDGE ( 'NONE', *, *, #119266, .T. ) ;
#94764=DIRECTION ( 'NONE',  ( 0.000000000000000000, 1.000000000000000000, 0.000000000000000000 ) ) ;
#94765=CARTESIAN_POINT ( 'NONE',  ( -11.64999999999999680, 2.500000000000000000, -2.757883832488650100 ) ) ;
#94766=CARTESIAN_POINT ( 'NONE',  ( -9.800000000000007816, 12.50000000000000000, -3.918623584224384615 ) ) ;
#94767=ORIENTED_EDGE ( 'NONE', *, *, #103073, .F. ) ;
#94768=EDGE_CURVE ( 'NONE', #37234, #6735, #115688, .T. ) ;
#94770=EDGE_CURVE ( 'NONE', #127507, #112646, #71899, .T. ) ;
#94771=EDGE_CURVE ( 'NONE', #43418, #65087, #34253, .T. ) ;
#94772=CONICAL_SURFACE ( 'NONE', #57114, 0.09999999999999982514, 0.003490658503988666988 ) ;
#94773=DIRECTION ( 'NONE',  ( 0.000000000000000000, 1.000000000000000000, 0.000000000000000000 ) ) ;
#94774=ORIENTED_EDGE ( 'NONE', *, *, #42177, .T. ) ;
#94775=VERTEX_POINT ( 'NONE', #78719 ) ;
#94776=VERTEX_POINT ( 'NONE', #11232 ) ;
#94777=ORIENTED_EDGE ( 'NONE', *, *, #2644, .F. ) ;
#94778=DIRECTION ( 'NONE',  ( 0.000000000000000000, 1.000000000000000000, 0.000000000000000000 ) ) ;
#94779=ADVANCED_FACE ( 'NONE', ( #79359 ), #15426, .T. ) ;
#94780=DIRECTION ( 'NONE',  ( 0.000000000000000000, 0.000000000000000000, 1.000000000000000000 ) ) ;
#94781=AXIS2_PLACEMENT_3D ( 'NONE', #111180, #115696, #122960 ) ;
#94782=FACE_OUTER_BOUND ( 'NONE', #55667, .T. ) ;
#94783=AXIS2_PLACEMENT_3D ( 'NONE', #79384, #49291, #118646 ) ;
#94784=EDGE_CURVE ( 'NONE', #60953, #124470, #61440, .T. ) ;
#94785=CARTESIAN_POINT ( 'NONE',  ( -8.100000000000013856, 2.500000000000000000, -0.3464101615137782364 ) ) ;
#94786=AXIS2_PLACEMENT_3D ( 'NONE', #12825, #10891, #102521 ) ;
#94787=EDGE_CURVE ( 'NONE', #40128, #96953, #9184, .T. ) ;
#94788=ORIENTED_EDGE ( 'NONE', *, *, #73819, .T. ) ;
#94789=DIRECTION ( 'NONE',  ( 0.000000000000000000, 1.000000000000000000, 0.000000000000000000 ) ) ;
#94790=ORIENTED_EDGE ( 'NONE', *, *, #116178, .F. ) ;
#94791=CARTESIAN_POINT ( 'NONE',  ( 87.50000000000001421, -3.974992050023849810, -6.359987280038161828 ) ) ;
#94792=DIRECTION ( 'NONE',  ( -0.000000000000000000, 1.000000000000000000, -0.000000000000000000 ) ) ;
#94793=CARTESIAN_POINT ( 'NONE',  ( 14.59999999999989484, 2.500000000000000000, -2.276824562219559311E-15 ) ) ;
#94794=CARTESIAN_POINT ( 'NONE',  ( 16.84158739990380482, -0.4722467112502861109, 5.802037699230406353 ) ) ;
#94795=CONICAL_SURFACE ( 'NONE', #98994, 0.09999999999999982514, 0.003490658503988666988 ) ;
#94796=VECTOR ( 'NONE', #47579, 1000.000000000000000 ) ;
#94797=AXIS2_PLACEMENT_3D ( 'NONE', #108696, #79252, #48490 ) ;
#94798=EDGE_LOOP ( 'NONE', ( #118465, #76188 ) ) ;
#94800=EDGE_LOOP ( 'NONE', ( #83571, #100516, #100655, #19420 ) ) ;
#94801=CARTESIAN_POINT ( 'NONE',  ( 7.899999999999924860, 2.500000000000000000, 4.430127018922196847 ) ) ;
#94802=CARTESIAN_POINT ( 'NONE',  ( 10.19999999999991402, 2.500000000000000000, 0.3464101615137735735 ) ) ;
#94803=CARTESIAN_POINT ( 'NONE',  ( -11.84999999999999609, 2.500000000000000000, 6.148780366869520897 ) ) ;
#94804=FACE_BOUND ( 'NONE', #79943, .T. ) ;
#94805=VECTOR ( 'NONE', #5005, 1000.000000000000000 ) ;
#94806=DIRECTION ( 'NONE',  ( 0.000000000000000000, 1.000000000000000000, 0.000000000000000000 ) ) ;
#94807=CARTESIAN_POINT ( 'NONE',  ( 3.549999999999942091, 2.500000000000000000, 2.411473670974873862 ) ) ;
#94808=DIRECTION ( 'NONE',  ( -0.000000000000000000, -1.000000000000000000, -0.000000000000000000 ) ) ;
#94809=AXIS2_PLACEMENT_3D ( 'NONE', #120718, #81446, #92539 ) ;
#94810=AXIS2_PLACEMENT_3D ( 'NONE', #26492, #16641, #96490 ) ;
#94811=AXIS2_PLACEMENT_3D ( 'NONE', #125453, #105820, #64600 ) ;
#94812=CARTESIAN_POINT ( 'NONE',  ( -1.900000000000034994, 12.50000000000000000, -4.741630453620016006 ) ) ;
#94813=DIRECTION ( 'NONE',  ( 0.000000000000000000, 0.000000000000000000, 1.000000000000000000 ) ) ;
#94814=AXIS2_PLACEMENT_3D ( 'NONE', #89367, #18683, #129314 ) ;
#94815=DIRECTION ( 'NONE',  ( 0.000000000000000000, 1.000000000000000000, 0.000000000000000000 ) ) ;
#94816=ORIENTED_EDGE ( 'NONE', *, *, #114389, .F. ) ;
#94817=FACE_OUTER_BOUND ( 'NONE', #49570, .T. ) ;
#94818=ORIENTED_EDGE ( 'NONE', *, *, #27506, .F. ) ;
#94819=VERTEX_POINT ( 'NONE', #41374 ) ;
#94820=EDGE_LOOP ( 'NONE', ( #55016, #93981, #77851, #25146 ) ) ;
#94822=CARTESIAN_POINT ( 'NONE',  ( 1.849999999999950573, 2.500000000000000000, -1.718653347947326049 ) ) ;
#94823=EDGE_CURVE ( 'NONE', #47303, #105454, #59293, .T. ) ;
#94824=FACE_BOUND ( 'NONE', #94458, .T. ) ;
#94826=EDGE_CURVE ( 'NONE', #22036, #8336, #88609, .T. ) ;
#94827=ADVANCED_FACE ( 'NONE', ( #61650 ), #104141, .T. ) ;
#94828=ORIENTED_EDGE ( 'NONE', *, *, #14338, .F. ) ;
#94829=CARTESIAN_POINT ( 'NONE',  ( 35.03103265460730142, 3.271231620377792026, 3.345711933278367578 ) ) ;
#94830=AXIS2_PLACEMENT_3D ( 'NONE', #20949, #90978, #1304 ) ;
#94831=DIRECTION ( 'NONE',  ( 0.000000000000000000, -0.000000000000000000, 1.000000000000000000 ) ) ;
#94832=ORIENTED_EDGE ( 'NONE', *, *, #116344, .F. ) ;
#94834=DIRECTION ( 'NONE',  ( -0.000000000000000000, 1.000000000000000000, -0.000000000000000000 ) ) ;
#94835=ADVANCED_FACE ( 'NONE', ( #34774 ), #11882, .T. ) ;
#94836=AXIS2_PLACEMENT_3D ( 'NONE', #53273, #93194, #84652 ) ;
#94837=CIRCLE ( 'NONE', #69704, 0.1000000000000002554 ) ;
#94838=VECTOR ( 'NONE', #67259, 1000.000000000000000 ) ;
#94839=AXIS2_PLACEMENT_3D ( 'NONE', #16763, #96618, #6940 ) ;
#94840=CIRCLE ( 'NONE', #32171, 0.09999999999999982514 ) ;
#94841=ORIENTED_EDGE ( 'NONE', *, *, #16176, .F. ) ;
#94842=FACE_OUTER_BOUND ( 'NONE', #27131, .T. ) ;
#94843=CARTESIAN_POINT ( 'NONE',  ( 4.599999999999940137, 12.50000000000000000, -4.265033745738164406 ) ) ;
#94844=CIRCLE ( 'NONE', #73912, 0.09999999999999982514 ) ;
#94845=AXIS2_PLACEMENT_3D ( 'NONE', #15156, #95043, #106144 ) ;
#94846=EDGE_LOOP ( 'NONE', ( #62498, #16570 ) ) ;
#94847=AXIS2_PLACEMENT_3D ( 'NONE', #37526, #117319, #27672 ) ;
#94848=CARTESIAN_POINT ( 'NONE',  ( 8.349999999999919709, 2.500000000000000000, -2.757883832488654097 ) ) ;
#94849=CARTESIAN_POINT ( 'NONE',  ( 12.09999999999990195, 12.50000000000000000, 0.7579135962115869374 ) ) ;
#94850=DIRECTION ( 'NONE',  ( 0.000000000000000000, 0.000000000000000000, 1.000000000000000000 ) ) ;
#94851=AXIS2_PLACEMENT_3D ( 'NONE', #96824, #28100, #117098 ) ;
#94852=EDGE_LOOP ( 'NONE', ( #7228, #108660 ) ) ;
#94853=ORIENTED_EDGE ( 'NONE', *, *, #43503, .F. ) ;
#94855=EDGE_CURVE ( 'NONE', #41716, #40814, #92375, .T. ) ;
#94856=VERTEX_POINT ( 'NONE', #123760 ) ;
#94857=DIRECTION ( 'NONE',  ( 0.000000000000000000, 0.000000000000000000, 1.000000000000000000 ) ) ;
#94858=DIRECTION ( 'NONE',  ( 0.000000000000000000, 1.000000000000000000, 0.000000000000000000 ) ) ;
#94859=ORIENTED_EDGE ( 'NONE', *, *, #125823, .T. ) ;
#94861=CARTESIAN_POINT ( 'NONE',  ( -8.750000000000012434, 2.500000000000000000, -5.802370205355744659 ) ) ;
#94862=DIRECTION ( 'NONE',  ( 0.000000000000000000, 0.000000000000000000, 1.000000000000000000 ) ) ;
#94863=FACE_OUTER_BOUND ( 'NONE', #119445, .T. ) ;
#94864=CARTESIAN_POINT ( 'NONE',  ( -5.400000000000024336, 2.500000000000000000, -3.537306695894649966 ) ) ;
#94865=AXIS2_PLACEMENT_3D ( 'NONE', #81284, #59067, #98984 ) ;
#94866=VERTEX_POINT ( 'NONE', #41999 ) ;
#94867=EDGE_LOOP ( 'NONE', ( #3628, #58086, #66817, #8052 ) ) ;
#94868=CARTESIAN_POINT ( 'NONE',  ( -2.700000000000031264, 12.50000000000000000, 4.611443907251934426 ) ) ;
#94869=ADVANCED_FACE ( 'NONE', ( #43943 ), #23777, .T. ) ;
#94870=CARTESIAN_POINT ( 'NONE',  ( 2.099999999999949463, 12.50000000000000000, -3.702399969078687292 ) ) ;
#94871=CARTESIAN_POINT ( 'NONE',  ( -0.6500000000000398792, 12.50000000000000000, -6.776507416713040577 ) ) ;
#94872=ORIENTED_EDGE ( 'NONE', *, *, #113301, .F. ) ;
#94873=ORIENTED_EDGE ( 'NONE', *, *, #77036, .T. ) ;
#94874=ORIENTED_EDGE ( 'NONE', *, *, #49018, .T. ) ;
#94875=DIRECTION ( 'NONE',  ( -0.000000000000000000, -1.000000000000000000, -0.000000000000000000 ) ) ;
#94876=VECTOR ( 'NONE', #95278, 1000.000000000000000 ) ;
#94877=AXIS2_PLACEMENT_3D ( 'NONE', #60402, #50543, #21090 ) ;
#94878=DIRECTION ( 'NONE',  ( 0.000000000000000000, 1.000000000000000000, 0.000000000000000000 ) ) ;
#94879=AXIS2_PLACEMENT_3D ( 'NONE', #54388, #72752, #24294 ) ;
#94880=CARTESIAN_POINT ( 'NONE',  ( 6.449999999999931788, 2.500000000000000000, 6.248780366869520542 ) ) ;
#94881=CARTESIAN_POINT ( 'NONE',  ( -10.65000000000000213, 12.50000000000000000, 6.148780366869520009 ) ) ;
#94882=FACE_OUTER_BOUND ( 'NONE', #75536, .T. ) ;
#94883=DIRECTION ( 'NONE',  ( -0.000000000000000000, 1.000000000000000000, -0.000000000000000000 ) ) ;
#94884=FACE_OUTER_BOUND ( 'NONE', #7771, .T. ) ;
#94885=DIRECTION ( 'NONE',  ( -0.000000000000000000, -1.000000000000000000, -0.000000000000000000 ) ) ;
#94886=EDGE_CURVE ( 'NONE', #125089, #26581, #40516, .T. ) ;
#94887=VECTOR ( 'NONE', #103187, 1000.000000000000000 ) ;
#94888=VECTOR ( 'NONE', #50797, 1000.000000000000000 ) ;
#94889=CARTESIAN_POINT ( 'NONE',  ( 14.34999999999989662, 12.50000000000000000, 2.511473670974873507 ) ) ;
#94890=AXIS2_PLACEMENT_3D ( 'NONE', #40303, #101799, #41603 ) ;
#94891=ORIENTED_EDGE ( 'NONE', *, *, #57268, .T. ) ;
#94892=VECTOR ( 'NONE', #57929, 1000.000000000000000 ) ;
#94893=DIRECTION ( 'NONE',  ( 0.000000000000000000, 0.000000000000000000, 1.000000000000000000 ) ) ;
#94894=VERTEX_POINT ( 'NONE', #84504 ) ;
#94895=EDGE_CURVE ( 'NONE', #44501, #3248, #67666, .T. ) ;
#94896=ORIENTED_EDGE ( 'NONE', *, *, #66308, .F. ) ;
#94897=DIRECTION ( 'NONE',  ( 0.000000000000000000, 1.000000000000000000, 0.000000000000000000 ) ) ;
#94898=DIRECTION ( 'NONE',  ( -4.274815082592931898E-19, -0.9999939076577903929, -0.003490651415223739937 ) ) ;
#94899=DIRECTION ( 'NONE',  ( 0.000000000000000000, -0.000000000000000000, 1.000000000000000000 ) ) ;
#94901=DIRECTION ( 'NONE',  ( -0.000000000000000000, 1.000000000000000000, -0.000000000000000000 ) ) ;
#94902=CIRCLE ( 'NONE', #107420, 0.1000000000000000472 ) ;
#94903=CARTESIAN_POINT ( 'NONE',  ( 2.049999999999948308, 12.50000000000000000, 6.560283801567334372 ) ) ;
#94904=AXIS2_PLACEMENT_3D ( 'NONE', #9189, #2571, #43185 ) ;
#94905=CONICAL_SURFACE ( 'NONE', #38494, 0.1000000000000002554, 0.003490658503988666988 ) ;
#94906=DIRECTION ( 'NONE',  ( -0.000000000000000000, 1.000000000000000000, -0.000000000000000000 ) ) ;
#94907=VERTEX_POINT ( 'NONE', #2057 ) ;
#94908=DIRECTION ( 'NONE',  ( -0.000000000000000000, 1.000000000000000000, -0.000000000000000000 ) ) ;
#94909=AXIS2_PLACEMENT_3D ( 'NONE', #129160, #19150, #79396 ) ;
#94910=CIRCLE ( 'NONE', #25961, 0.1000000000000000056 ) ;
#94911=CARTESIAN_POINT ( 'NONE',  ( -5.800000000000022027, 2.500000000000000000, -4.430127018922202176 ) ) ;
#94912=ORIENTED_EDGE ( 'NONE', *, *, #67128, .F. ) ;
#94913=ORIENTED_EDGE ( 'NONE', *, *, #90693, .T. ) ;
#94914=EDGE_CURVE ( 'NONE', #18083, #60727, #17480, .T. ) ;
#94915=ORIENTED_EDGE ( 'NONE', *, *, #112627, .T. ) ;
#94916=ORIENTED_EDGE ( 'NONE', *, *, #87515, .F. ) ;
#94917=CARTESIAN_POINT ( 'NONE',  ( 9.599999999999914380, 2.500000000000000000, -5.022947341949754119 ) ) ;
#94918=CARTESIAN_POINT ( 'NONE',  ( -3.750000000000031086, 12.50000000000000000, -5.802370205355749988 ) ) ;
#94919=EDGE_CURVE ( 'NONE', #113079, #100019, #101134, .T. ) ;
#94920=DIRECTION ( 'NONE',  ( 0.000000000000000000, 0.000000000000000000, 1.000000000000000000 ) ) ;
#94921=DIRECTION ( 'NONE',  ( 0.000000000000000000, 0.000000000000000000, 1.000000000000000000 ) ) ;
#94922=VECTOR ( 'NONE', #63355, 1000.000000000000000 ) ;
#94923=DIRECTION ( 'NONE',  ( 0.000000000000000000, -0.9999939076577903929, 0.003490651415223739937 ) ) ;
#94925=DIRECTION ( 'NONE',  ( -0.000000000000000000, 1.000000000000000000, -0.000000000000000000 ) ) ;
#94926=CONICAL_SURFACE ( 'NONE', #53173, 0.09999999999999982514, 0.003490658503988666988 ) ;
#94927=EDGE_CURVE ( 'NONE', #92392, #117253, #57212, .T. ) ;
#94928=VECTOR ( 'NONE', #43686, 1000.000000000000000 ) ;
#94929=ADVANCED_FACE ( 'NONE', ( #94304 ), #111358, .T. ) ;
#94930=ADVANCED_FACE ( 'NONE', ( #73379 ), #90659, .T. ) ;
#94931=DIRECTION ( 'NONE',  ( 0.000000000000000000, 1.000000000000000000, 0.000000000000000000 ) ) ;
#94932=EDGE_CURVE ( 'NONE', #100183, #104358, #22377, .T. ) ;
#94934=EDGE_LOOP ( 'NONE', ( #9774, #116566, #26217, #59766 ) ) ;
#94935=CIRCLE ( 'NONE', #2999, 0.06509327318403745899 ) ;
#94936=CIRCLE ( 'NONE', #38519, 0.06509327318403745899 ) ;
#94937=VECTOR ( 'NONE', #98454, 1000.000000000000000 ) ;
#94938=ORIENTED_EDGE ( 'NONE', *, *, #96541, .F. ) ;
#94939=CIRCLE ( 'NONE', #63548, 0.06509327318403745899 ) ;
#94940=EDGE_CURVE ( 'NONE', #89101, #99935, #103501, .T. ) ;
#94941=ORIENTED_EDGE ( 'NONE', *, *, #5831, .T. ) ;
#94942=CARTESIAN_POINT ( 'NONE',  ( 4.149999999999939959, 12.50000000000000000, -6.495190528383302464 ) ) ;
#94943=ADVANCED_FACE ( 'NONE', ( #122498 ), #4966, .T. ) ;
#94944=EDGE_CURVE ( 'NONE', #18483, #54425, #113650, .T. ) ;
#94945=DIRECTION ( 'NONE',  ( 0.000000000000000000, 1.000000000000000000, 0.000000000000000000 ) ) ;
#94946=PLANE ( 'NONE',  #64 ) ;
#94947=CIRCLE ( 'NONE', #63554, 0.1000000000000002554 ) ;
#94948=EDGE_CURVE ( 'NONE', #92599, #29210, #72750, .T. ) ;
#94949=AXIS2_PLACEMENT_3D ( 'NONE', #66851, #35482, #76687 ) ;
#94950=CIRCLE ( 'NONE', #53193, 0.06509327318403745899 ) ;
#94951=EDGE_CURVE ( 'NONE', #40542, #12969, #84397, .T. ) ;
#94952=VECTOR ( 'NONE', #58224, 1000.000000000000000 ) ;
#94953=ORIENTED_EDGE ( 'NONE', *, *, #13443, .T. ) ;
#94954=DIRECTION ( 'NONE',  ( -0.000000000000000000, 1.000000000000000000, -0.000000000000000000 ) ) ;
#94955=FACE_OUTER_BOUND ( 'NONE', #50983, .T. ) ;
#94956=CARTESIAN_POINT ( 'NONE',  ( 3.749999999999975131, 12.50000000000000000, 6.495190528383297135 ) ) ;
#94957=CARTESIAN_POINT ( 'NONE',  ( -10.40000000000000213, 2.500000000000000000, -0.6928203230275541413 ) ) ;
#94958=CARTESIAN_POINT ( 'NONE',  ( 10.19999999999991402, 2.500000000000000000, 0.3464101615137735735 ) ) ;
#94959=EDGE_CURVE ( 'NONE', #36386, #11332, #105333, .T. ) ;
#94960=ORIENTED_EDGE ( 'NONE', *, *, #116067, .F. ) ;
#94961=LINE ( 'NONE', #83208, #127199 ) ;
#94962=ORIENTED_EDGE ( 'NONE', *, *, #29798, .F. ) ;
#94963=ORIENTED_EDGE ( 'NONE', *, *, #320, .F. ) ;
#94964=VERTEX_POINT ( 'NONE', #7208 ) ;
#94965=CARTESIAN_POINT ( 'NONE',  ( -2.050000000000033129, 2.500000000000000000, 2.165063509461097713 ) ) ;
#94966=FACE_BOUND ( 'NONE', #1656, .T. ) ;
#94967=DIRECTION ( 'NONE',  ( -0.000000000000000000, -1.000000000000000000, -0.000000000000000000 ) ) ;
#94968=FACE_OUTER_BOUND ( 'NONE', #116039, .T. ) ;
#94969=DIRECTION ( 'NONE',  ( 0.000000000000000000, 0.000000000000000000, 1.000000000000000000 ) ) ;
#94970=EDGE_LOOP ( 'NONE', ( #6557, #79110, #37789, #38175 ) ) ;
#94971=DIRECTION ( 'NONE',  ( 0.000000000000000000, 1.000000000000000000, 0.000000000000000000 ) ) ;
#94972=CARTESIAN_POINT ( 'NONE',  ( 10.84999999999990905, 2.500000000000000000, 1.472243186433545459 ) ) ;
#94973=FACE_OUTER_BOUND ( 'NONE', #13567, .T. ) ;
#94974=CARTESIAN_POINT ( 'NONE',  ( 9.599999999999917932, 12.50000000000000000, 0.6928203230275494784 ) ) ;
#94975=ORIENTED_EDGE ( 'NONE', *, *, #21504, .F. ) ;
#94976=AXIS2_PLACEMENT_3D ( 'NONE', #5945, #43967, #66168 ) ;
#94977=AXIS2_PLACEMENT_3D ( 'NONE', #109294, #60845, #100746 ) ;
#94978=DIRECTION ( 'NONE',  ( 0.000000000000000000, 1.000000000000000000, 0.000000000000000000 ) ) ;
#94979=DIRECTION ( 'NONE',  ( 0.000000000000000000, 1.000000000000000000, 0.000000000000000000 ) ) ;
#94980=VERTEX_POINT ( 'NONE', #26231 ) ;
#94981=CARTESIAN_POINT ( 'NONE',  ( -7.100000000000014744, 12.50000000000000000, 4.395220292106234439 ) ) ;
#94982=ORIENTED_EDGE ( 'NONE', *, *, #109076, .T. ) ;
#94983=FACE_BOUND ( 'NONE', #42286, .T. ) ;
#94984=CARTESIAN_POINT ( 'NONE',  ( 10.59999999999990905, 12.50000000000000000, 3.983716857408420076 ) ) ;
#94985=VECTOR ( 'NONE', #23144, 1000.000000000000000 ) ;
#94986=ADVANCED_FACE ( 'NONE', ( #77260 ), #19563, .T. ) ;
#94987=ORIENTED_EDGE ( 'NONE', *, *, #104064, .F. ) ;
#94988=CARTESIAN_POINT ( 'NONE',  ( -10.00000000000000355, 12.50000000000000000, -0.6928203230275541413 ) ) ;
#94989=CARTESIAN_POINT ( 'NONE',  ( 3.549999999999940314, 2.500000000000000000, 6.841600689897072485 ) ) ;
#94990=EDGE_CURVE ( 'NONE', #73565, #42572, #82267, .T. ) ;
#94991=VERTEX_POINT ( 'NONE', #65493 ) ;
#94992=EDGE_LOOP ( 'NONE', ( #126066, #9403, #3209, #112487 ) ) ;
#94994=ORIENTED_EDGE ( 'NONE', *, *, #98927, .F. ) ;
#94995=DIRECTION ( 'NONE',  ( 0.000000000000000000, 0.000000000000000000, 1.000000000000000000 ) ) ;
#94996=DIRECTION ( 'NONE',  ( 0.000000000000000000, 1.000000000000000000, 0.000000000000000000 ) ) ;
#94997=EDGE_CURVE ( 'NONE', #123263, #87864, #104757, .T. ) ;
#94998=AXIS2_PLACEMENT_3D ( 'NONE', #24298, #3998, #104145 ) ;
#94999=AXIS2_PLACEMENT_3D ( 'NONE', #1427, #102842, #13168 ) ;
#95000=CARTESIAN_POINT ( 'NONE',  ( 14.14999999999989733, 2.500000000000000000, 2.957883832488649389 ) ) ;
#95001=DIRECTION ( 'NONE',  ( 0.000000000000000000, 1.000000000000000000, 0.000000000000000000 ) ) ;
#95002=DIRECTION ( 'NONE',  ( 0.000000000000000000, 0.000000000000000000, 1.000000000000000000 ) ) ;
#95003=AXIS2_PLACEMENT_3D ( 'NONE', #80686, #121242, #30947 ) ;
#95005=CIRCLE ( 'NONE', #32337, 0.06509327318403745899 ) ;
#95006=ORIENTED_EDGE ( 'NONE', *, *, #82237, .T. ) ;
#95007=ORIENTED_EDGE ( 'NONE', *, *, #16278, .F. ) ;
#95008=CARTESIAN_POINT ( 'NONE',  ( 8.549999999999922551, 2.500000000000000000, 2.611473670974873151 ) ) ;
#95009=DIRECTION ( 'NONE',  ( 0.000000000000000000, 0.000000000000000000, -1.000000000000000000 ) ) ;
#95010=DIRECTION ( 'NONE',  ( 0.000000000000000000, 1.000000000000000000, 0.000000000000000000 ) ) ;
#95011=CARTESIAN_POINT ( 'NONE',  ( 11.84999999999990372, 12.50000000000000000, -6.213873640053564351 ) ) ;
#95012=EDGE_LOOP ( 'NONE', ( #29387, #54573 ) ) ;
#95013=ORIENTED_EDGE ( 'NONE', *, *, #119973, .F. ) ;
#95014=FACE_BOUND ( 'NONE', #37587, .T. ) ;
#95015=ORIENTED_EDGE ( 'NONE', *, *, #96121, .F. ) ;
#95016=DIRECTION ( 'NONE',  ( -0.000000000000000000, 1.000000000000000000, -0.000000000000000000 ) ) ;
#95017=DIRECTION ( 'NONE',  ( 0.000000000000000000, 1.000000000000000000, 0.000000000000000000 ) ) ;
#95018=EDGE_LOOP ( 'NONE', ( #3760, #112067, #50773, #42450 ) ) ;
#95019=DIRECTION ( 'NONE',  ( 0.000000000000000000, 0.000000000000000000, 1.000000000000000000 ) ) ;
#95020=FACE_OUTER_BOUND ( 'NONE', #65814, .T. ) ;
#95021=FACE_OUTER_BOUND ( 'NONE', #87520, .T. ) ;
#95022=VECTOR ( 'NONE', #29540, 1000.000000000000000 ) ;
#95023=DIRECTION ( 'NONE',  ( -0.000000000000000000, 1.000000000000000000, -0.000000000000000000 ) ) ;
#95024=CIRCLE ( 'NONE', #72042, 0.06509327318403741736 ) ;
#95025=DIRECTION ( 'NONE',  ( 0.000000000000000000, 0.000000000000000000, 1.000000000000000000 ) ) ;
#95026=DIRECTION ( 'NONE',  ( 0.000000000000000000, 0.000000000000000000, 1.000000000000000000 ) ) ;
#95027=CIRCLE ( 'NONE', #23925, 0.06509327318403745899 ) ;
#95029=CARTESIAN_POINT ( 'NONE',  ( 3.549999999999944755, 2.500000000000000000, -6.941600689897077459 ) ) ;
#95030=CARTESIAN_POINT ( 'NONE',  ( 10.64999999999991331, 12.50000000000000000, 6.841600689897072485 ) ) ;
#95032=ORIENTED_EDGE ( 'NONE', *, *, #60584, .F. ) ;
#95033=ORIENTED_EDGE ( 'NONE', *, *, #116075, .T. ) ;
#95034=DIRECTION ( 'NONE',  ( 0.000000000000000000, -0.9999939076577903929, 0.003490651415223739937 ) ) ;
#95035=EDGE_LOOP ( 'NONE', ( #106520, #113639, #79306, #14307 ) ) ;
#95036=CARTESIAN_POINT ( 'NONE',  ( -1.250000000000037970, 2.500000000000000000, 2.757883832488649656 ) ) ;
#95037=ORIENTED_EDGE ( 'NONE', *, *, #111123, .F. ) ;
#95038=EDGE_LOOP ( 'NONE', ( #71839, #92305 ) ) ;
#95039=ORIENTED_EDGE ( 'NONE', *, *, #89075, .F. ) ;
#95040=PLANE ( 'NONE',  #8098 ) ;
#95041=AXIS2_PLACEMENT_3D ( 'NONE', #119055, #126944, #28093 ) ;
#95042=AXIS2_PLACEMENT_3D ( 'NONE', #34653, #105301, #16246 ) ;
#95043=DIRECTION ( 'NONE',  ( -0.000000000000000000, 1.000000000000000000, -0.000000000000000000 ) ) ;
#95045=CARTESIAN_POINT ( 'NONE',  ( -3.550000000000030909, 12.50000000000000000, -6.841600689897078702 ) ) ;
#95047=AXIS2_PLACEMENT_3D ( 'NONE', #35832, #75743, #26020 ) ;
#95048=EDGE_CURVE ( 'NONE', #42483, #5536, #69734, .T. ) ;
#95050=ORIENTED_EDGE ( 'NONE', *, *, #75531, .T. ) ;
#95051=EDGE_CURVE ( 'NONE', #50689, #8757, #46759, .T. ) ;
#95052=DIRECTION ( 'NONE',  ( -4.274815082592931898E-19, -0.9999939076577903929, -0.003490651415223739937 ) ) ;
#95053=VERTEX_POINT ( 'NONE', #25560 ) ;
#95054=ORIENTED_EDGE ( 'NONE', *, *, #81891, .F. ) ;
#95055=ORIENTED_EDGE ( 'NONE', *, *, #8599, .F. ) ;
#95056=DIRECTION ( 'NONE',  ( -4.274815082592931898E-19, -0.9999939076577903929, -0.003490651415223739937 ) ) ;
#95057=ORIENTED_EDGE ( 'NONE', *, *, #47438, .T. ) ;
#95058=EDGE_CURVE ( 'NONE', #28288, #48604, #73939, .T. ) ;
#95059=ORIENTED_EDGE ( 'NONE', *, *, #26493, .F. ) ;
#95060=ORIENTED_EDGE ( 'NONE', *, *, #78079, .F. ) ;
#95061=CIRCLE ( 'NONE', #126354, 0.1000000000000000472 ) ;
#95063=DIRECTION ( 'NONE',  ( 0.000000000000000000, 0.000000000000000000, -1.000000000000000000 ) ) ;
#95064=DIRECTION ( 'NONE',  ( 0.000000000000000000, 0.000000000000000000, -1.000000000000000000 ) ) ;
#95065=DIRECTION ( 'NONE',  ( 0.000000000000000000, 0.000000000000000000, 1.000000000000000000 ) ) ;
#95066=DIRECTION ( 'NONE',  ( -4.274815082592931898E-19, -0.9999939076577903929, -0.003490651415223739937 ) ) ;
#95067=DIRECTION ( 'NONE',  ( -0.000000000000000000, 1.000000000000000000, -0.000000000000000000 ) ) ;
#95068=ORIENTED_EDGE ( 'NONE', *, *, #45921, .F. ) ;
#95069=CARTESIAN_POINT ( 'NONE',  ( -0.8500000000000386136, 12.50000000000000000, 1.537336459617582918 ) ) ;
#95070=AXIS2_PLACEMENT_3D ( 'NONE', #70376, #100477, #128686 ) ;
#95071=EDGE_LOOP ( 'NONE', ( #83743, #122453 ) ) ;
#95072=CARTESIAN_POINT ( 'NONE',  ( 10.84999999999990905, 12.50000000000000000, 2.165063509461097713 ) ) ;
#95073=VERTEX_POINT ( 'NONE', #17679 ) ;
#95074=CARTESIAN_POINT ( 'NONE',  ( 3.549999999999942979, 2.500000000000000000, 1.818653347947321475 ) ) ;
#95075=ORIENTED_EDGE ( 'NONE', *, *, #4777, .T. ) ;
#95076=ORIENTED_EDGE ( 'NONE', *, *, #88989, .F. ) ;
#95077=CARTESIAN_POINT ( 'NONE',  ( -0.4000000000000331624, 2.500000000000000000, 0.1000000000000000056 ) ) ;
#95078=CARTESIAN_POINT ( 'NONE',  ( -1.850000000000033840, 12.50000000000000000, 6.148780366869520897 ) ) ;
#95079=EDGE_CURVE ( 'NONE', #96322, #2505, #24937, .T. ) ;
#95080=DIRECTION ( 'NONE',  ( -0.000000000000000000, 1.000000000000000000, -0.000000000000000000 ) ) ;
#95081=DIRECTION ( 'NONE',  ( 0.000000000000000000, -0.9999939076577903929, 0.003490651415223739937 ) ) ;
#95082=ORIENTED_EDGE ( 'NONE', *, *, #2145, .F. ) ;
#95083=CARTESIAN_POINT ( 'NONE',  ( -4.999999999999990230, 2.500000000000000000, -4.330127018922201643 ) ) ;
#95084=DIRECTION ( 'NONE',  ( 0.000000000000000000, 0.000000000000000000, 1.000000000000000000 ) ) ;
#95085=EDGE_CURVE ( 'NONE', #77033, #121438, #5066, .T. ) ;
#95086=FACE_OUTER_BOUND ( 'NONE', #22728, .T. ) ;
#95087=DIRECTION ( 'NONE',  ( 0.000000000000000000, 0.000000000000000000, 1.000000000000000000 ) ) ;
#95089=DIRECTION ( 'NONE',  ( -0.000000000000000000, -1.000000000000000000, -0.000000000000000000 ) ) ;
#95090=ORIENTED_EDGE ( 'NONE', *, *, #103648, .T. ) ;
#95091=CIRCLE ( 'NONE', #28190, 0.06509327318403745899 ) ;
#95092=AXIS2_PLACEMENT_3D ( 'NONE', #18035, #18687, #69728 ) ;
#95093=ORIENTED_EDGE ( 'NONE', *, *, #106648, .T. ) ;
#95094=EDGE_CURVE ( 'NONE', #91010, #384, #103286, .T. ) ;
#95095=EDGE_CURVE ( 'NONE', #94262, #28931, #35409, .T. ) ;
#95096=AXIS2_PLACEMENT_3D ( 'NONE', #103871, #89693, #119796 ) ;
#95097=EDGE_CURVE ( 'NONE', #76936, #83004, #63572, .T. ) ;
#95098=ORIENTED_EDGE ( 'NONE', *, *, #113680, .F. ) ;
#95099=CIRCLE ( 'NONE', #38680, 0.1000000000000002554 ) ;
#95100=CARTESIAN_POINT ( 'NONE',  ( 12.29999999999990479, 12.50000000000000000, -3.918623584224389056 ) ) ;
#95101=FACE_OUTER_BOUND ( 'NONE', #106180, .T. ) ;
#95102=EDGE_CURVE ( 'NONE', #110215, #997, #37347, .T. ) ;
#95104=DIRECTION ( 'NONE',  ( -0.000000000000000000, -1.000000000000000000, -0.000000000000000000 ) ) ;
#95105=DIRECTION ( 'NONE',  ( 0.000000000000000000, 1.000000000000000000, 0.000000000000000000 ) ) ;
#95106=DIRECTION ( 'NONE',  ( -0.000000000000000000, -1.000000000000000000, -0.000000000000000000 ) ) ;
#95107=CARTESIAN_POINT ( 'NONE',  ( 3.349999999999944578, 2.500000000000000000, -5.702370205355749455 ) ) ;
#95108=ORIENTED_EDGE ( 'NONE', *, *, #48276, .F. ) ;
#95109=EDGE_CURVE ( 'NONE', #23072, #87541, #107358, .T. ) ;
#95110=CIRCLE ( 'NONE', #26061, 0.09999999999999982514 ) ;
#95111=DIRECTION ( 'NONE',  ( 0.000000000000000000, 1.000000000000000000, 0.000000000000000000 ) ) ;
#95112=DIRECTION ( 'NONE',  ( 0.000000000000000000, 1.000000000000000000, 0.000000000000000000 ) ) ;
#95113=AXIS2_PLACEMENT_3D ( 'NONE', #40191, #38263, #108902 ) ;
#95114=ORIENTED_EDGE ( 'NONE', *, *, #71633, .F. ) ;
#95115=AXIS2_PLACEMENT_3D ( 'NONE', #116587, #26294, #105499 ) ;
#95116=CARTESIAN_POINT ( 'NONE',  ( -0.8500000000000390576, 12.50000000000000000, -2.165063509461101710 ) ) ;
#95117=CARTESIAN_POINT ( 'NONE',  ( 105.5000000000000142, 0.000000000000000000, 2.000000000000000000 ) ) ;
#95119=CONICAL_SURFACE ( 'NONE', #99328, 0.09999999999999999167, 0.003490658503988666988 ) ;
#95120=VECTOR ( 'NONE', #76509, 1000.000000000000000 ) ;
#95121=EDGE_LOOP ( 'NONE', ( #99299, #96831, #20902, #36935 ) ) ;
#95122=AXIS2_PLACEMENT_3D ( 'NONE', #87314, #39553, #89901 ) ;
#95123=DIRECTION ( 'NONE',  ( -0.000000000000000000, 1.000000000000000000, -0.000000000000000000 ) ) ;
#95124=ORIENTED_EDGE ( 'NONE', *, *, #112206, .F. ) ;
#95125=CARTESIAN_POINT ( 'NONE',  ( 4.999999999999971578, 12.50000000000000000, -2.276824562219559311E-15 ) ) ;
#95126=CARTESIAN_POINT ( 'NONE',  ( -0.8000000000000315747, 12.50000000000000000, 0.000000000000000000 ) ) ;
#95128=B_SPLINE_CURVE_WITH_KNOTS ( 'NONE', 3,
 ( #116542, #26883, #66790, #17015, #107374, #19650, #100143, #68735, #128326, #38662, #78582, #118475, #90963, #89031, #11091, #61520 ),
 .UNSPECIFIED., .F., .F.,
 ( 4, 2, 2, 2, 2, 2, 2, 4 ),
 ( 0.000000000000000000, 0.003502803217043994836, 0.007005606434087989672, 0.008757008042609990342, 0.01050840965113199015, 0.01225981125965399168, 0.01313551206391498985, 0.01401121286817599149 ),
 .UNSPECIFIED. ) ;
#95129=ORIENTED_EDGE ( 'NONE', *, *, #42855, .T. ) ;
#95130=CIRCLE ( 'NONE', #86713, 0.1000000000000000472 ) ;
#95131=AXIS2_PLACEMENT_3D ( 'NONE', #117343, #36259, #127216 ) ;
#95132=LINE ( 'NONE', #123927, #86485 ) ;
#95133=DIRECTION ( 'NONE',  ( -0.000000000000000000, 1.000000000000000000, -0.000000000000000000 ) ) ;
#95134=CIRCLE ( 'NONE', #97275, 0.06509327318403745899 ) ;
#95135=ORIENTED_EDGE ( 'NONE', *, *, #62860, .T. ) ;
#95136=CARTESIAN_POINT ( 'NONE',  ( -4.350000000000023626, 2.500000000000000000, 6.248780366869521430 ) ) ;
#95137=EDGE_CURVE ( 'NONE', #118811, #60113, #5911, .T. ) ;
#95138=ORIENTED_EDGE ( 'NONE', *, *, #22406, .T. ) ;
#95139=EDGE_LOOP ( 'NONE', ( #77664, #109799 ) ) ;
#95140=CARTESIAN_POINT ( 'NONE',  ( 7.299999999999924327, 2.500000000000000000, 0.3464101615137735735 ) ) ;
#95141=DIRECTION ( 'NONE',  ( -0.000000000000000000, 1.000000000000000000, -0.000000000000000000 ) ) ;
#95142=ORIENTED_EDGE ( 'NONE', *, *, #99345, .F. ) ;
#95143=CARTESIAN_POINT ( 'NONE',  ( 9.549999999999915445, 12.50000000000000000, 6.495190528383297135 ) ) ;
#95144=LINE ( 'NONE', #16556, #8741 ) ;
#95145=CIRCLE ( 'NONE', #107666, 0.06509327318403745899 ) ;
#95146=VERTEX_POINT ( 'NONE', #36051 ) ;
#95147=EDGE_CURVE ( 'NONE', #28723, #107807, #55257, .T. ) ;
#95148=DIRECTION ( 'NONE',  ( 0.000000000000000000, 1.000000000000000000, 0.000000000000000000 ) ) ;
#95149=DIRECTION ( 'NONE',  ( 0.000000000000000000, -0.000000000000000000, 1.000000000000000000 ) ) ;
#95150=DIRECTION ( 'NONE',  ( 0.000000000000000000, 0.000000000000000000, 1.000000000000000000 ) ) ;
#95151=DIRECTION ( 'NONE',  ( 0.000000000000000000, 0.000000000000000000, 1.000000000000000000 ) ) ;
#95152=DIRECTION ( 'NONE',  ( 0.000000000000000000, 1.000000000000000000, 0.000000000000000000 ) ) ;
#95153=CONICAL_SURFACE ( 'NONE', #5349, 0.1000000000000002554, 0.003490658503988666988 ) ;
#95154=CARTESIAN_POINT ( 'NONE',  ( -11.05000000000000071, 2.500000000000000000, 6.741600689897071952 ) ) ;
#95155=AXIS2_PLACEMENT_3D ( 'NONE', #61859, #2261, #5482 ) ;
#95156=AXIS2_PLACEMENT_3D ( 'NONE', #10302, #20767, #59429 ) ;
#95157=EDGE_LOOP ( 'NONE', ( #27163, #8677 ) ) ;
#95158=ORIENTED_EDGE ( 'NONE', *, *, #45561, .T. ) ;
#95159=EDGE_LOOP ( 'NONE', ( #53757, #3418 ) ) ;
#95160=ORIENTED_EDGE ( 'NONE', *, *, #31523, .T. ) ;
#95161=CARTESIAN_POINT ( 'NONE',  ( 59.86274543073836440, 3.775833904478943737, 4.995381933851997580 ) ) ;
#95163=DIRECTION ( 'NONE',  ( 0.000000000000000000, -0.9999939076577903929, 0.003490651415223739937 ) ) ;
#95164=ORIENTED_EDGE ( 'NONE', *, *, #87762, .F. ) ;
#95165=FACE_BOUND ( 'NONE', #58899, .T. ) ;
#95166=CARTESIAN_POINT ( 'NONE',  ( -1.850000000000033840, 2.500000000000000000, 2.611473670974873151 ) ) ;
#95167=LINE ( 'NONE', #8062, #87744 ) ;
#95168=CIRCLE ( 'NONE', #38762, 0.06509327318403745899 ) ;
#95169=DIRECTION ( 'NONE',  ( 0.000000000000000000, -0.000000000000000000, 1.000000000000000000 ) ) ;
#95170=FACE_OUTER_BOUND ( 'NONE', #111127, .T. ) ;
#95171=CONICAL_SURFACE ( 'NONE', #74242, 0.1000000000000000472, 0.003490658503988666988 ) ;
#95172=CARTESIAN_POINT ( 'NONE',  ( -1.650000000000034772, 12.50000000000000000, 5.737276932171707422 ) ) ;
#95173=CARTESIAN_POINT ( 'NONE',  ( -11.64999999999999680, 2.500000000000000000, 2.165063509461097713 ) ) ;
#95174=DIRECTION ( 'NONE',  ( -0.000000000000000000, 1.000000000000000000, -0.000000000000000000 ) ) ;
#95175=DIRECTION ( 'NONE',  ( 0.000000000000000000, 0.000000000000000000, 1.000000000000000000 ) ) ;
#95176=CARTESIAN_POINT ( 'NONE',  ( 4.999999999999971578, 12.50000000000000000, -0.06509327318403970719 ) ) ;
#95177=DIRECTION ( 'NONE',  ( 0.000000000000000000, 1.000000000000000000, 0.000000000000000000 ) ) ;
#95178=EDGE_CURVE ( 'NONE', #25799, #52300, #82368, .T. ) ;
#95179=CIRCLE ( 'NONE', #40826, 0.06509327318403745899 ) ;
#95180=ORIENTED_EDGE ( 'NONE', *, *, #9685, .T. ) ;
#95181=ORIENTED_EDGE ( 'NONE', *, *, #1700, .F. ) ;
#95182=CIRCLE ( 'NONE', #51376, 0.1000000000000002554 ) ;
#95183=VERTEX_POINT ( 'NONE', #8497 ) ;
#95184=ORIENTED_EDGE ( 'NONE', *, *, #29390, .F. ) ;
#95185=DIRECTION ( 'NONE',  ( 0.000000000000000000, 1.000000000000000000, 0.000000000000000000 ) ) ;
#95186=EDGE_LOOP ( 'NONE', ( #128009, #15254, #115081, #28510 ) ) ;
#95187=CARTESIAN_POINT ( 'NONE',  ( 3.349999999999945466, 2.500000000000000000, -2.165063509461101710 ) ) ;
#95188=ORIENTED_EDGE ( 'NONE', *, *, #11830, .T. ) ;
#95189=VERTEX_POINT ( 'NONE', #80499 ) ;
#95190=LINE ( 'NONE', #46735, #62611 ) ;
#95191=EDGE_CURVE ( 'NONE', #20105, #81996, #42660, .T. ) ;
#95192=CONICAL_SURFACE ( 'NONE', #38782, 0.1000000000000002554, 0.003490658503988666988 ) ;
#95193=CARTESIAN_POINT ( 'NONE',  ( 10.06913504587715202, -2.500000000000000444, 8.158951466338434599 ) ) ;
#95194=DIRECTION ( 'NONE',  ( 0.000000000000000000, 1.000000000000000000, 0.000000000000000000 ) ) ;
#95195=CARTESIAN_POINT ( 'NONE',  ( 5.199999999999935341, 12.50000000000000000, -3.983716857408426293 ) ) ;
#95196=DIRECTION ( 'NONE',  ( -0.000000000000000000, 1.000000000000000000, -0.000000000000000000 ) ) ;
#95197=EDGE_CURVE ( 'NONE', #114600, #108081, #108645, .T. ) ;
#95198=EDGE_CURVE ( 'NONE', #104829, #83303, #124207, .T. ) ;
#95199=CONICAL_SURFACE ( 'NONE', #65845, 0.09999999999999982514, 0.003490658503988666988 ) ;
#95200=ORIENTED_EDGE ( 'NONE', *, *, #97501, .T. ) ;
#95201=ORIENTED_EDGE ( 'NONE', *, *, #29012, .F. ) ;
#95202=CIRCLE ( 'NONE', #78497, 0.06509327318403745899 ) ;
#95203=ORIENTED_EDGE ( 'NONE', *, *, #122718, .F. ) ;
#95204=DIRECTION ( 'NONE',  ( 0.000000000000000000, 1.000000000000000000, 0.000000000000000000 ) ) ;
#95205=ORIENTED_EDGE ( 'NONE', *, *, #8764, .F. ) ;
#95206=EDGE_CURVE ( 'NONE', #11701, #50102, #107486, .T. ) ;
#95207=AXIS2_PLACEMENT_3D ( 'NONE', #44862, #105041, #95246 ) ;
#95208=CARTESIAN_POINT ( 'NONE',  ( 7.499999999999927169, 2.500000000000000000, -4.922947341949753586 ) ) ;
#95209=ORIENTED_EDGE ( 'NONE', *, *, #59469, .F. ) ;
#95210=EDGE_CURVE ( 'NONE', #24001, #121148, #80301, .T. ) ;
#95211=ORIENTED_EDGE ( 'NONE', *, *, #54864, .F. ) ;
#95212=DIRECTION ( 'NONE',  ( -0.000000000000000000, 1.000000000000000000, -0.000000000000000000 ) ) ;
#95213=AXIS2_PLACEMENT_3D ( 'NONE', #8583, #47261, #19049 ) ;
#95214=AXIS2_PLACEMENT_3D ( 'NONE', #31922, #120301, #111092 ) ;
#95215=AXIS2_PLACEMENT_3D ( 'NONE', #125170, #74140, #24391 ) ;
#95216=DIRECTION ( 'NONE',  ( 0.000000000000000000, 1.000000000000000000, 0.000000000000000000 ) ) ;
#95217=FACE_OUTER_BOUND ( 'NONE', #18592, .T. ) ;
#95219=CONICAL_SURFACE ( 'NONE', #78513, 0.1000000000000002554, 0.003490658503988666988 ) ;
#95220=DIRECTION ( 'NONE',  ( 0.000000000000000000, 1.000000000000000000, 0.000000000000000000 ) ) ;
#95221=ORIENTED_EDGE ( 'NONE', *, *, #52949, .F. ) ;
#95222=CARTESIAN_POINT ( 'NONE',  ( 7.899999999999924860, 2.500000000000000000, -4.330127018922201643 ) ) ;
#95224=AXIS2_PLACEMENT_3D ( 'NONE', #67622, #107568, #17885 ) ;
#95225=VERTEX_POINT ( 'NONE', #119118 ) ;
#95226=CARTESIAN_POINT ( 'NONE',  ( 14.59999999999989484, 12.50000000000000000, -2.276824562219559311E-15 ) ) ;
#95227=CONICAL_SURFACE ( 'NONE', #38819, 0.09999999999999982514, 0.003490658503988666988 ) ;
#95228=ORIENTED_EDGE ( 'NONE', *, *, #112519, .T. ) ;
#95229=CARTESIAN_POINT ( 'NONE',  ( 12.49999999999990230, 2.500000000000000000, -0.7928203230275542301 ) ) ;
#95230=CARTESIAN_POINT ( 'NONE',  ( -8.749999999999976907, 2.500000000000000000, -6.495190528383297135 ) ) ;
#95231=AXIS2_PLACEMENT_3D ( 'NONE', #28930, #77375, #58393 ) ;
#95232=ORIENTED_EDGE ( 'NONE', *, *, #68585, .T. ) ;
#95233=LINE ( 'NONE', #4888, #29979 ) ;
#95234=FACE_OUTER_BOUND ( 'NONE', #101577, .T. ) ;
#95236=DIRECTION ( 'NONE',  ( 0.000000000000000000, 0.000000000000000000, 1.000000000000000000 ) ) ;
#95237=ADVANCED_FACE ( 'NONE', ( #69356 ), #109291, .T. ) ;
#95238=DIRECTION ( 'NONE',  ( -0.000000000000000000, 1.000000000000000000, -0.000000000000000000 ) ) ;
#95239=ORIENTED_EDGE ( 'NONE', *, *, #66404, .F. ) ;
#95240=ORIENTED_EDGE ( 'NONE', *, *, #38524, .F. ) ;
#95241=VERTEX_POINT ( 'NONE', #78569 ) ;
#95242=FACE_OUTER_BOUND ( 'NONE', #122625, .T. ) ;
#95243=CARTESIAN_POINT ( 'NONE',  ( -9.150000000000009237, 12.50000000000000000, 1.472243186433545459 ) ) ;
#95245=AXIS2_PLACEMENT_3D ( 'NONE', #59617, #119150, #20312 ) ;
#95246=DIRECTION ( 'NONE',  ( 0.000000000000000000, 0.000000000000000000, -1.000000000000000000 ) ) ;
#95247=ADVANCED_FACE ( 'NONE', ( #108000 ), #57310, .T. ) ;
#95248=CARTESIAN_POINT ( 'NONE',  ( 11.69999999999990514, 2.500000000000000000, -0.1000000000000022815 ) ) ;
#95249=DIRECTION ( 'NONE',  ( -0.000000000000000000, 1.000000000000000000, -0.000000000000000000 ) ) ;
#95251=AXIS2_PLACEMENT_3D ( 'NONE', #13209, #1462, #102260 ) ;
#95252=EDGE_CURVE ( 'NONE', #48345, #49639, #67766, .T. ) ;
#95253=CIRCLE ( 'NONE', #105716, 0.06509327318403745899 ) ;
#95254=ADVANCED_FACE ( 'NONE', ( #19634 ), #92826, .T. ) ;
#95255=ORIENTED_EDGE ( 'NONE', *, *, #87927, .T. ) ;
#95256=CIRCLE ( 'NONE', #74321, 0.1000000000000002554 ) ;
#95257=CARTESIAN_POINT ( 'NONE',  ( 10.39999999999991509, 2.500000000000000000, 0.7928203230275495672 ) ) ;
#95258=EDGE_LOOP ( 'NONE', ( #49512, #113367 ) ) ;
#95259=ADVANCED_FACE ( 'NONE', ( #90275 ), #88343, .T. ) ;
#95260=CARTESIAN_POINT ( 'NONE',  ( -0.6500000000000398792, 2.500000000000000000, -6.841600689897078702 ) ) ;
#95261=DIRECTION ( 'NONE',  ( -0.000000000000000000, 1.000000000000000000, -0.000000000000000000 ) ) ;
#95262=DIRECTION ( 'NONE',  ( 0.000000000000000000, 1.000000000000000000, 0.000000000000000000 ) ) ;
#95263=ORIENTED_EDGE ( 'NONE', *, *, #106012, .T. ) ;
#95264=EDGE_CURVE ( 'NONE', #32613, #108881, #50374, .T. ) ;
#95265=AXIS2_PLACEMENT_3D ( 'NONE', #112525, #113151, #42500 ) ;
#95266=ADVANCED_FACE ( 'NONE', ( #118461 ), #53107, .T. ) ;
#95267=VECTOR ( 'NONE', #72476, 1000.000000000000000 ) ;
#95268=LINE ( 'NONE', #65130, #20006 ) ;
#95269=CARTESIAN_POINT ( 'NONE',  ( -12.29999999999999538, 2.500000000000000000, 4.576537180435972019 ) ) ;
#95270=ORIENTED_EDGE ( 'NONE', *, *, #4794, .T. ) ;
#95271=FACE_OUTER_BOUND ( 'NONE', #100505, .T. ) ;
#95272=CIRCLE ( 'NONE', #45105, 0.1000000000000002554 ) ;
#95273=AXIS2_PLACEMENT_3D ( 'NONE', #83893, #84548, #75360 ) ;
#95274=ORIENTED_EDGE ( 'NONE', *, *, #96237, .T. ) ;
#95275=ORIENTED_EDGE ( 'NONE', *, *, #71733, .T. ) ;
#95276=CARTESIAN_POINT ( 'NONE',  ( -9.800000000000004263, 2.500000000000000000, 3.883716857408420431 ) ) ;
#95277=ORIENTED_EDGE ( 'NONE', *, *, #65352, .F. ) ;
#95278=DIRECTION ( 'NONE',  ( 0.000000000000000000, -0.9999939076577903929, 0.003490651415223739937 ) ) ;
#95279=CARTESIAN_POINT ( 'NONE',  ( -8.100000000000013856, 12.50000000000000000, 0.3464101615137736845 ) ) ;
#95280=CARTESIAN_POINT ( 'NONE',  ( -0.8500000000000382805, 2.500000000000000000, -5.702370205355749455 ) ) ;
#95281=ORIENTED_EDGE ( 'NONE', *, *, #21941, .F. ) ;
#95282=FACE_BOUND ( 'NONE', #22497, .T. ) ;
#95283=CARTESIAN_POINT ( 'NONE',  ( -6.249999999999981348, 12.50000000000000000, 2.165063509461097713 ) ) ;
#95285=PLANE ( 'NONE',  #15161 ) ;
#95286=DIRECTION ( 'NONE',  ( 0.000000000000000000, 0.000000000000000000, -1.000000000000000000 ) ) ;
#95287=VERTEX_POINT ( 'NONE', #89660 ) ;
#95288=AXIS2_PLACEMENT_3D ( 'NONE', #36261, #16585, #27704 ) ;
#95289=ORIENTED_EDGE ( 'NONE', *, *, #71253, .T. ) ;
#95290=VECTOR ( 'NONE', #112799, 1000.000000000000000 ) ;
#95291=ORIENTED_EDGE ( 'NONE', *, *, #71560, .T. ) ;
#95292=FACE_OUTER_BOUND ( 'NONE', #45448, .T. ) ;
#95293=LINE ( 'NONE', #84816, #97986 ) ;
#95295=DIRECTION ( 'NONE',  ( 0.000000000000000000, 0.000000000000000000, -1.000000000000000000 ) ) ;
#95296=FACE_BOUND ( 'NONE', #50494, .T. ) ;
#95297=ORIENTED_EDGE ( 'NONE', *, *, #115005, .F. ) ;
#95300=LINE ( 'NONE', #5602, #23013 ) ;
#95301=EDGE_CURVE ( 'NONE', #73914, #67694, #111687, .T. ) ;
#95302=CARTESIAN_POINT ( 'NONE',  ( -1.700000000000034817, 2.500000000000000000, -2.385244779468109755E-15 ) ) ;
#95303=CARTESIAN_POINT ( 'NONE',  ( 10.44999999999991402, 2.500000000000000000, 6.495190528383297135 ) ) ;
#95304=CIRCLE ( 'NONE', #128778, 0.09999999999999999167 ) ;
#95305=CARTESIAN_POINT ( 'NONE',  ( 2.949999999999946887, 2.500000000000000000, -6.395190528383301931 ) ) ;
#95306=CARTESIAN_POINT ( 'NONE',  ( -13.14999999999999147, 12.50000000000000000, -1.818653347947323917 ) ) ;
#95307=CARTESIAN_POINT ( 'NONE',  ( -6.050000000000020250, 2.500000000000000000, -2.511473670974877948 ) ) ;
#95308=AXIS2_PLACEMENT_3D ( 'NONE', #36098, #16416, #56364 ) ;
#95309=FACE_OUTER_BOUND ( 'NONE', #120014, .T. ) ;
#95310=CONICAL_SURFACE ( 'NONE', #61878, 0.1000000000000000472, 0.003490658503988666988 ) ;
#95311=VERTEX_POINT ( 'NONE', #6329 ) ;
#95312=ORIENTED_EDGE ( 'NONE', *, *, #92290, .F. ) ;
#95313=VERTEX_POINT ( 'NONE', #96653 ) ;
#95314=VERTEX_POINT ( 'NONE', #87483 ) ;
#95315=AXIS2_PLACEMENT_3D ( 'NONE', #25364, #93488, #5724 ) ;
#95316=ORIENTED_EDGE ( 'NONE', *, *, #35673, .F. ) ;
#95317=FACE_OUTER_BOUND ( 'NONE', #97642, .T. ) ;
#95318=DIRECTION ( 'NONE',  ( 0.000000000000000000, 0.000000000000000000, -1.000000000000000000 ) ) ;
#95319=ORIENTED_EDGE ( 'NONE', *, *, #6711, .T. ) ;
#95320=FACE_BOUND ( 'NONE', #1146, .T. ) ;
#95321=CARTESIAN_POINT ( 'NONE',  ( 4.799999999999935874, 12.50000000000000000, 3.983716857408420964 ) ) ;
#95323=VERTEX_POINT ( 'NONE', #95390 ) ;
#95324=DIRECTION ( 'NONE',  ( -0.000000000000000000, 1.000000000000000000, -0.000000000000000000 ) ) ;
#95326=CARTESIAN_POINT ( 'NONE',  ( -1.900000000000034994, 2.500000000000000000, -4.676537180435978769 ) ) ;
#95327=AXIS2_PLACEMENT_3D ( 'NONE', #93563, #3251, #91623 ) ;
#95328=VERTEX_POINT ( 'NONE', #77668 ) ;
#95329=CARTESIAN_POINT ( 'NONE',  ( 5.799999999999933209, 2.500000000000000000, -2.385244779468109755E-15 ) ) ;
#95330=ORIENTED_EDGE ( 'NONE', *, *, #25456, .T. ) ;
#95332=ORIENTED_EDGE ( 'NONE', *, *, #15962, .F. ) ;
#95333=VERTEX_POINT ( 'NONE', #106497 ) ;
#95334=CARTESIAN_POINT ( 'NONE',  ( -1.850000000000033396, 2.500000000000000000, -2.611473670974877592 ) ) ;
#95335=CARTESIAN_POINT ( 'NONE',  ( -6.249999999999984901, 2.500000000000000000, -6.495190528383302464 ) ) ;
#95336=CIRCLE ( 'NONE', #5524, 0.1000000000000002554 ) ;
#95337=DIRECTION ( 'NONE',  ( -0.000000000000000000, -1.000000000000000000, -0.000000000000000000 ) ) ;
#95339=CARTESIAN_POINT ( 'NONE',  ( 11.74779829703379974, 2.500000000000000000, -7.682567037525008580 ) ) ;
#95340=CIRCLE ( 'NONE', #38935, 0.1000000000000002554 ) ;
#95341=VECTOR ( 'NONE', #118002, 1000.000000000000000 ) ;
#95342=EDGE_CURVE ( 'NONE', #14399, #115596, #109545, .T. ) ;
#95343=CARTESIAN_POINT ( 'NONE',  ( 12.09999999999990550, 2.500000000000000000, -3.637306695894650055 ) ) ;
#95344=AXIS2_PLACEMENT_3D ( 'NONE', #44433, #73252, #122366 ) ;
#95345=DIRECTION ( 'NONE',  ( 0.000000000000000000, 0.000000000000000000, 1.000000000000000000 ) ) ;
#95347=PLANE ( 'NONE',  #71820 ) ;
#95348=EDGE_CURVE ( 'NONE', #80050, #20142, #71984, .T. ) ;
#95350=ADVANCED_FACE ( 'NONE', ( #65265 ), #56096, .T. ) ;
#95351=EDGE_LOOP ( 'NONE', ( #15612, #104300 ) ) ;
#95352=FACE_OUTER_BOUND ( 'NONE', #5850, .T. ) ;
#95353=CIRCLE ( 'NONE', #128832, 0.06509327318403745899 ) ;
#95354=ORIENTED_EDGE ( 'NONE', *, *, #12933, .F. ) ;
#95355=AXIS2_PLACEMENT_3D ( 'NONE', #79894, #78630, #71348 ) ;
#95356=AXIS2_PLACEMENT_3D ( 'NONE', #114949, #25274, #73736 ) ;
#95357=ORIENTED_EDGE ( 'NONE', *, *, #60518, .T. ) ;
#95358=CARTESIAN_POINT ( 'NONE',  ( 12.89999999999990266, 2.500000000000000000, -3.637306695894650055 ) ) ;
#95359=CARTESIAN_POINT ( 'NONE',  ( 11.89999999999990798, 2.500000000000000000, 3.983716857408420964 ) ) ;
#95360=EDGE_CURVE ( 'NONE', #39771, #86684, #107785, .T. ) ;
#95361=EDGE_CURVE ( 'NONE', #101786, #91215, #65918, .T. ) ;
#95362=LINE ( 'NONE', #43704, #109479 ) ;
#95363=CARTESIAN_POINT ( 'NONE',  ( -7.300000000000016698, 2.500000000000000000, -0.4464101615137783252 ) ) ;
#95364=ADVANCED_FACE ( 'NONE', ( #46950 ), #117572, .T. ) ;
#95365=ORIENTED_EDGE ( 'NONE', *, *, #99912, .F. ) ;
#95366=ORIENTED_EDGE ( 'NONE', *, *, #89892, .F. ) ;
#95367=CARTESIAN_POINT ( 'NONE',  ( 2.699999999999946443, 2.500000000000000000, -4.083716857408426826 ) ) ;
#95368=CARTESIAN_POINT ( 'NONE',  ( 11.84999999999990372, 2.500000000000000000, -6.841600689897078702 ) ) ;
#95369=CARTESIAN_POINT ( 'NONE',  ( -12.09999999999999609, 2.500000000000000000, -5.022947341949751454 ) ) ;
#95370=ORIENTED_EDGE ( 'NONE', *, *, #91088, .T. ) ;
#95371=ORIENTED_EDGE ( 'NONE', *, *, #87778, .F. ) ;
#95372=CARTESIAN_POINT ( 'NONE',  ( 11.84999999999990372, 12.50000000000000000, 1.818653347947321475 ) ) ;
#95373=ORIENTED_EDGE ( 'NONE', *, *, #87828, .T. ) ;
#95374=DIRECTION ( 'NONE',  ( 0.000000000000000000, 0.000000000000000000, 1.000000000000000000 ) ) ;
#95375=CARTESIAN_POINT ( 'NONE',  ( 5.799999999999934985, 2.500000000000000000, -4.230127018922201998 ) ) ;
#95376=ORIENTED_EDGE ( 'NONE', *, *, #88546, .F. ) ;
#95377=CARTESIAN_POINT ( 'NONE',  ( -4.999999999999986677, 2.500000000000000000, -2.276824562219559311E-15 ) ) ;
#95378=CARTESIAN_POINT ( 'NONE',  ( -1.250000000000037970, 12.50000000000000000, 7.253104124594885960 ) ) ;
#95379=CARTESIAN_POINT ( 'NONE',  ( -11.44999999999999929, 2.500000000000000000, -6.148780366869522673 ) ) ;
#95380=CARTESIAN_POINT ( 'NONE',  ( -0.2000000000000412836, 12.50000000000000000, 4.676537180435972552 ) ) ;
#95381=ORIENTED_EDGE ( 'NONE', *, *, #12301, .F. ) ;
#95382=DIRECTION ( 'NONE',  ( -0.000000000000000000, -1.000000000000000000, -0.000000000000000000 ) ) ;
#95383=AXIS2_PLACEMENT_3D ( 'NONE', #10019, #42730, #121903 ) ;
#95384=CIRCLE ( 'NONE', #112196, 0.1000000000000002554 ) ;
#95385=FACE_OUTER_BOUND ( 'NONE', #112197, .T. ) ;
#95386=ORIENTED_EDGE ( 'NONE', *, *, #27353, .F. ) ;
#95387=ORIENTED_EDGE ( 'NONE', *, *, #91409, .F. ) ;
#95389=DIRECTION ( 'NONE',  ( -0.000000000000000000, 1.000000000000000000, -0.000000000000000000 ) ) ;
#95390=CARTESIAN_POINT ( 'NONE',  ( 10.39999999999991154, 2.500000000000000000, -3.537306695894649966 ) ) ;
#95391=FACE_OUTER_BOUND ( 'NONE', #110548, .T. ) ;
#95392=CARTESIAN_POINT ( 'NONE',  ( -0.6500000000000403233, 2.500000000000000000, 1.718653347947321386 ) ) ;
#95393=CONICAL_SURFACE ( 'NONE', #126791, 0.1000000000000002554, 0.003490658503988666988 ) ;
#95394=DIRECTION ( 'NONE',  ( 0.000000000000000000, -0.000000000000000000, 1.000000000000000000 ) ) ;
#95395=DIRECTION ( 'NONE',  ( -0.000000000000000000, 1.000000000000000000, -0.000000000000000000 ) ) ;
#95396=DIRECTION ( 'NONE',  ( 0.000000000000000000, 0.000000000000000000, -1.000000000000000000 ) ) ;
#95397=CARTESIAN_POINT ( 'NONE',  ( 5.849999999999933920, 2.500000000000000000, -2.757883832488654097 ) ) ;
#95398=DIRECTION ( 'NONE',  ( 0.000000000000000000, -0.9999939076577903929, 0.003490651415223739937 ) ) ;
#95399=EDGE_CURVE ( 'NONE', #18200, #68464, #126788, .T. ) ;
#95400=EDGE_CURVE ( 'NONE', #111304, #45268, #34344, .T. ) ;
#95401=EDGE_CURVE ( 'NONE', #7829, #117308, #23870, .T. ) ;
#95402=DIRECTION ( 'NONE',  ( 0.000000000000000000, 1.000000000000000000, 0.000000000000000000 ) ) ;
#95403=VECTOR ( 'NONE', #25051, 1000.000000000000000 ) ;
#95404=AXIS2_PLACEMENT_3D ( 'NONE', #24301, #23653, #3999 ) ;
#95406=EDGE_LOOP ( 'NONE', ( #22920, #22904, #21709, #39838 ) ) ;
#95407=EDGE_CURVE ( 'NONE', #64709, #62921, #49007, .T. ) ;
#95408=ORIENTED_EDGE ( 'NONE', *, *, #19990, .T. ) ;
#95409=EDGE_CURVE ( 'NONE', #96334, #4778, #75735, .T. ) ;
#95410=DIRECTION ( 'NONE',  ( -0.000000000000000000, 1.000000000000000000, -0.000000000000000000 ) ) ;
#95411=FACE_OUTER_BOUND ( 'NONE', #17659, .T. ) ;
#95412=EDGE_CURVE ( 'NONE', #115890, #62546, #120007, .T. ) ;
#95413=ORIENTED_EDGE ( 'NONE', *, *, #47287, .F. ) ;
#95414=EDGE_CURVE ( 'NONE', #83814, #73789, #65708, .T. ) ;
#95415=CARTESIAN_POINT ( 'NONE',  ( -14.99999999999994671, 2.500000000000000000, 0.000000000000000000 ) ) ;
#95416=EDGE_CURVE ( 'NONE', #19273, #8444, #128076, .T. ) ;
#95417=DIRECTION ( 'NONE',  ( -0.000000000000000000, 1.000000000000000000, -0.000000000000000000 ) ) ;
#95418=FACE_OUTER_BOUND ( 'NONE', #85239, .T. ) ;
#95419=ORIENTED_EDGE ( 'NONE', *, *, #49906, .F. ) ;
#95420=AXIS2_PLACEMENT_3D ( 'NONE', #28697, #58797, #9033 ) ;
#95421=ADVANCED_FACE ( 'NONE', ( #38423 ), #7637, .T. ) ;
#95422=CARTESIAN_POINT ( 'NONE',  ( 9.149999999999920419, 2.500000000000000000, -7.288010851410854585 ) ) ;
#95423=VERTEX_POINT ( 'NONE', #116299 ) ;
#95424=AXIS2_PLACEMENT_3D ( 'NONE', #80155, #8175, #88006 ) ;
#95425=AXIS2_PLACEMENT_3D ( 'NONE', #57888, #78170, #8119 ) ;
#95426=ORIENTED_EDGE ( 'NONE', *, *, #61960, .F. ) ;
#95427=VERTEX_POINT ( 'NONE', #26653 ) ;
#95428=VERTEX_POINT ( 'NONE', #66558 ) ;
#95429=CARTESIAN_POINT ( 'NONE',  ( -8.100000000000013856, 2.500000000000000000, -0.4464101615137782142 ) ) ;
#95431=CIRCLE ( 'NONE', #107950, 0.06509327318403745899 ) ;
#95432=DIRECTION ( 'NONE',  ( 0.000000000000000000, 0.000000000000000000, 1.000000000000000000 ) ) ;
#95433=CARTESIAN_POINT ( 'NONE',  ( 11.24999999999991118, 12.50000000000000000, -2.857883832488653741 ) ) ;
#95434=VECTOR ( 'NONE', #97720, 1000.000000000000000 ) ;
#95435=DIRECTION ( 'NONE',  ( 0.000000000000000000, 0.000000000000000000, 1.000000000000000000 ) ) ;
#95436=ORIENTED_EDGE ( 'NONE', *, *, #23968, .F. ) ;
#95437=CONICAL_SURFACE ( 'NONE', #36861, 0.09999999999999982514, 0.003490658503988666988 ) ;
#95438=CARTESIAN_POINT ( 'NONE',  ( -13.14999999999999147, 2.500000000000000000, 2.411473670974877415 ) ) ;
#95439=ORIENTED_EDGE ( 'NONE', *, *, #16883, .T. ) ;
#95440=LINE ( 'NONE', #45701, #126971 ) ;
#95441=CARTESIAN_POINT ( 'NONE',  ( 16.04820284657690621, -2.500000000000000444, -6.585610460626504903 ) ) ;
#95442=DIRECTION ( 'NONE',  ( 0.000000000000000000, 0.000000000000000000, -1.000000000000000000 ) ) ;
#95443=PLANE ( 'NONE',  #111218 ) ;
#95444=CONICAL_SURFACE ( 'NONE', #39041, 0.09999999999999982514, 0.003490658503988666988 ) ;
#95445=ORIENTED_EDGE ( 'NONE', *, *, #77619, .F. ) ;
#95446=AXIS2_PLACEMENT_3D ( 'NONE', #12905, #24052, #72513 ) ;
#95447=CIRCLE ( 'NONE', #47330, 0.1000000000000002554 ) ;
#95448=VERTEX_POINT ( 'NONE', #16795 ) ;
#95449=ORIENTED_EDGE ( 'NONE', *, *, #76925, .T. ) ;
#95450=DIRECTION ( 'NONE',  ( -4.274815082592931898E-19, -0.9999939076577903929, -0.003490651415223739937 ) ) ;
#95451=FACE_OUTER_BOUND ( 'NONE', #89524, .T. ) ;
#95452=FACE_OUTER_BOUND ( 'NONE', #67972, .T. ) ;
#95453=FACE_BOUND ( 'NONE', #1717, .T. ) ;
#95454=LINE ( 'NONE', #45716, #57708 ) ;
#95455=FACE_OUTER_BOUND ( 'NONE', #87858, .T. ) ;
#95456=CARTESIAN_POINT ( 'NONE',  ( 7.949999999999925571, 12.50000000000000000, -6.430097255199264339 ) ) ;
#95457=CARTESIAN_POINT ( 'NONE',  ( -4.119968255444916849E-14, 2.500000000000000000, 3.637306695894644726 ) ) ;
#95458=ADVANCED_FACE ( 'NONE', ( #56720 ), #43419, .T. ) ;
#95459=CARTESIAN_POINT ( 'NONE',  ( 8.349999999999919709, 2.500000000000000000, 6.595190528383296780 ) ) ;
#95460=CARTESIAN_POINT ( 'NONE',  ( 1.899999999999951283, 2.500000000000000000, 0.2464101615137736789 ) ) ;
#95461=DIRECTION ( 'NONE',  ( 0.000000000000000000, -0.000000000000000000, 1.000000000000000000 ) ) ;
#95462=CARTESIAN_POINT ( 'NONE',  ( -3.100000000000028955, 2.500000000000000000, 4.676537180435972552 ) ) ;
#95463=ORIENTED_EDGE ( 'NONE', *, *, #50314, .T. ) ;
#95464=EDGE_LOOP ( 'NONE', ( #83590, #85663, #41055, #73305 ) ) ;
#95465=ORIENTED_EDGE ( 'NONE', *, *, #33736, .F. ) ;
#95466=ORIENTED_EDGE ( 'NONE', *, *, #106024, .T. ) ;
#95467=ADVANCED_FACE ( 'NONE', ( #20702 ), #49100, .T. ) ;
#95468=DIRECTION ( 'NONE',  ( -4.274815082592931898E-19, -0.9999939076577903929, -0.003490651415223739937 ) ) ;
#95469=FACE_BOUND ( 'NONE', #60563, .T. ) ;
#95470=DIRECTION ( 'NONE',  ( 0.000000000000000000, 1.000000000000000000, 0.000000000000000000 ) ) ;
#95471=AXIS2_PLACEMENT_3D ( 'NONE', #109346, #99545, #1321 ) ;
#95472=CONICAL_SURFACE ( 'NONE', #93329, 0.09999999999999982514, 0.003490658503988666988 ) ;
#95473=ORIENTED_EDGE ( 'NONE', *, *, #73202, .F. ) ;
#95474=DIRECTION ( 'NONE',  ( -4.274815082592931898E-19, -0.9999939076577903929, -0.003490651415223739937 ) ) ;
#95475=DIRECTION ( 'NONE',  ( 0.000000000000000000, 1.000000000000000000, 0.000000000000000000 ) ) ;
#95476=VERTEX_POINT ( 'NONE', #69795 ) ;
#95477=CARTESIAN_POINT ( 'NONE',  ( -12.09999999999999609, 2.500000000000000000, 0.5928203230275536084 ) ) ;
#95478=FACE_OUTER_BOUND ( 'NONE', #87848, .T. ) ;
#95479=AXIS2_PLACEMENT_3D ( 'NONE', #37955, #95589, #47139 ) ;
#95480=VECTOR ( 'NONE', #121869, 1000.000000000000000 ) ;
#95481=ORIENTED_EDGE ( 'NONE', *, *, #48165, .T. ) ;
#95482=DIRECTION ( 'NONE',  ( -4.274815082592931898E-19, -0.9999939076577903929, -0.003490651415223739937 ) ) ;
#95483=LINE ( 'NONE', #5793, #9961 ) ;
#95484=CONICAL_SURFACE ( 'NONE', #39082, 0.1000000000000002554, 0.003490658503988666988 ) ;
#95485=CIRCLE ( 'NONE', #47383, 0.09999999999999999167 ) ;
#95486=CIRCLE ( 'NONE', #105952, 0.09999999999999982514 ) ;
#95487=VERTEX_POINT ( 'NONE', #68497 ) ;
#95488=AXIS2_PLACEMENT_3D ( 'NONE', #45424, #85334, #34973 ) ;
#95489=EDGE_CURVE ( 'NONE', #122496, #43147, #99269, .T. ) ;
#95490=CARTESIAN_POINT ( 'NONE',  ( 7.899999999999924860, 2.500000000000000000, -3.637306695894650055 ) ) ;
#95491=CARTESIAN_POINT ( 'NONE',  ( -13.54999999999999005, 12.50000000000000000, 2.511473670974877503 ) ) ;
#95492=ORIENTED_EDGE ( 'NONE', *, *, #19716, .T. ) ;
#95493=DIRECTION ( 'NONE',  ( 0.000000000000000000, -0.9999939076577903929, 0.003490651415223739937 ) ) ;
#95494=ORIENTED_EDGE ( 'NONE', *, *, #108528, .F. ) ;
#95495=ORIENTED_EDGE ( 'NONE', *, *, #95361, .T. ) ;
#95496=FACE_OUTER_BOUND ( 'NONE', #62294, .T. ) ;
#95497=EDGE_CURVE ( 'NONE', #78788, #22205, #40351, .T. ) ;
#95498=ORIENTED_EDGE ( 'NONE', *, *, #56789, .F. ) ;
#95499=LINE ( 'NONE', #86306, #17734 ) ;
#95500=DIRECTION ( 'NONE',  ( 0.000000000000000000, -0.9999939076577903929, 0.003490651415223739937 ) ) ;
#95501=VERTEX_POINT ( 'NONE', #9588 ) ;
#95502=DIRECTION ( 'NONE',  ( 0.000000000000000000, 0.000000000000000000, -1.000000000000000000 ) ) ;
#95503=DIRECTION ( 'NONE',  ( 0.000000000000000000, 0.000000000000000000, 1.000000000000000000 ) ) ;
#95504=DIRECTION ( 'NONE',  ( 0.000000000000000000, 0.000000000000000000, -1.000000000000000000 ) ) ;
#95505=EDGE_CURVE ( 'NONE', #127904, #99888, #10821, .T. ) ;
#95506=ADVANCED_FACE ( 'NONE', ( #119527 ), #122254, .T. ) ;
#95507=CARTESIAN_POINT ( 'NONE',  ( -3.550000000000027800, 2.500000000000000000, 6.148780366869520009 ) ) ;
#95508=EDGE_CURVE ( 'NONE', #81743, #82923, #95061, .T. ) ;
#95509=DIRECTION ( 'NONE',  ( 0.000000000000000000, 0.000000000000000000, 1.000000000000000000 ) ) ;
#95510=EDGE_CURVE ( 'NONE', #62380, #29817, #38643, .T. ) ;
#95511=AXIS2_PLACEMENT_3D ( 'NONE', #25288, #54755, #75684 ) ;
#95512=ADVANCED_FACE ( 'NONE', ( #70443 ), #60002, .T. ) ;
#95513=CARTESIAN_POINT ( 'NONE',  ( 8.349999999999919709, 2.500000000000000000, 5.802370205355744659 ) ) ;
#95514=CIRCLE ( 'NONE', #28619, 0.1000000000000002554 ) ;
#95515=AXIS2_PLACEMENT_3D ( 'NONE', #9214, #106757, #119166 ) ;
#95516=ORIENTED_EDGE ( 'NONE', *, *, #75847, .F. ) ;
#95517=EDGE_LOOP ( 'NONE', ( #31228, #15639 ) ) ;
#95518=FACE_OUTER_BOUND ( 'NONE', #16863, .T. ) ;
#95519=AXIS2_PLACEMENT_3D ( 'NONE', #19793, #66932, #77418 ) ;
#95520=DIRECTION ( 'NONE',  ( 0.000000000000000000, 1.000000000000000000, 0.000000000000000000 ) ) ;
#95521=CARTESIAN_POINT ( 'NONE',  ( 11.44999999999991047, 12.50000000000000000, 6.083687093685482772 ) ) ;
#95522=VERTEX_POINT ( 'NONE', #120830 ) ;
#95523=ORIENTED_EDGE ( 'NONE', *, *, #86705, .F. ) ;
#95524=ORIENTED_EDGE ( 'NONE', *, *, #45463, .T. ) ;
#95525=ADVANCED_FACE ( 'NONE', ( #128745 ), #17674, .T. ) ;
#95526=CARTESIAN_POINT ( 'NONE',  ( -3.100000000000028955, 2.500000000000000000, 4.676537180435972552 ) ) ;
#95527=CONICAL_SURFACE ( 'NONE', #39112, 0.1000000000000000056, 0.003490658503988666988 ) ;
#95528=CIRCLE ( 'NONE', #108030, 0.1000000000000002554 ) ;
#95529=ADVANCED_FACE ( 'NONE', ( #10235 ), #18753, .T. ) ;
#95530=CARTESIAN_POINT ( 'NONE',  ( -1.450000000000035039, 2.500000000000000000, -6.941600689897077459 ) ) ;
#95531=EDGE_CURVE ( 'NONE', #94071, #105417, #8921, .T. ) ;
#95532=DIRECTION ( 'NONE',  ( -4.274815082592931898E-19, -0.9999939076577903929, -0.003490651415223739937 ) ) ;
#95533=CIRCLE ( 'NONE', #112259, 0.1000000000000002554 ) ;
#95535=CARTESIAN_POINT ( 'NONE',  ( -0.8500000000000382805, 2.500000000000000000, -7.188010851410854052 ) ) ;
#95536=FACE_OUTER_BOUND ( 'NONE', #56186, .T. ) ;
#95537=CARTESIAN_POINT ( 'NONE',  ( 12.29999999999990301, 2.500000000000000000, -0.3464101615137782364 ) ) ;
#95538=DIRECTION ( 'NONE',  ( -4.274815082592931898E-19, -0.9999939076577903929, -0.003490651415223739937 ) ) ;
#95539=DIRECTION ( 'NONE',  ( 0.000000000000000000, 0.000000000000000000, 1.000000000000000000 ) ) ;
#95540=FACE_OUTER_BOUND ( 'NONE', #5597, .T. ) ;
#95542=VECTOR ( 'NONE', #359, 1000.000000000000000 ) ;
#95543=AXIS2_PLACEMENT_3D ( 'NONE', #23688, #55720, #5961 ) ;
#95544=CARTESIAN_POINT ( 'NONE',  ( -6.250000000000015987, 2.500000000000000000, 5.802370205355744659 ) ) ;
#95545=EDGE_LOOP ( 'NONE', ( #70782, #55328, #69973, #109231 ) ) ;
#95546=ORIENTED_EDGE ( 'NONE', *, *, #20199, .T. ) ;
#95547=DIRECTION ( 'NONE',  ( -0.000000000000000000, -1.000000000000000000, -0.000000000000000000 ) ) ;
#95548=CARTESIAN_POINT ( 'NONE',  ( 9.999999999999911182, 2.500000000000000000, 4.922947341949748257 ) ) ;
#95549=CARTESIAN_POINT ( 'NONE',  ( 13.29999999999989946, 12.50000000000000000, -2.385244779468109755E-15 ) ) ;
#95550=LINE ( 'NONE', #85077, #127781 ) ;
#95551=CARTESIAN_POINT ( 'NONE',  ( -2.900000000000029665, 12.50000000000000000, 4.330127018922196314 ) ) ;
#95552=DIRECTION ( 'NONE',  ( 0.000000000000000000, -0.9999939076577903929, 0.003490651415223739937 ) ) ;
#95553=PLANE ( 'NONE',  #109621 ) ;
#95554=VERTEX_POINT ( 'NONE', #118247 ) ;
#95555=CARTESIAN_POINT ( 'NONE',  ( 13.34999999999990017, 2.500000000000000000, 2.757883832488649656 ) ) ;
#95556=AXIS2_PLACEMENT_3D ( 'NONE', #55425, #62676, #75063 ) ;
#95557=EDGE_CURVE ( 'NONE', #66518, #110514, #29243, .T. ) ;
#95558=LINE ( 'NONE', #106021, #58280 ) ;
#95559=VERTEX_POINT ( 'NONE', #109048 ) ;
#95560=EDGE_LOOP ( 'NONE', ( #51140, #48090, #105378, #128187 ) ) ;
#95561=EDGE_CURVE ( 'NONE', #21383, #32164, #19388, .T. ) ;
#95563=ADVANCED_FACE ( 'NONE', ( #79615 ), #29872, .T. ) ;
#95564=ORIENTED_EDGE ( 'NONE', *, *, #105107, .T. ) ;
#95565=CARTESIAN_POINT ( 'NONE',  ( -1.250000000000035749, 12.50000000000000000, -2.857883832488653741 ) ) ;
#95566=DIRECTION ( 'NONE',  ( 0.000000000000000000, 1.000000000000000000, 0.000000000000000000 ) ) ;
#95567=EDGE_CURVE ( 'NONE', #124646, #13639, #13466, .T. ) ;
#95568=AXIS2_PLACEMENT_3D ( 'NONE', #18226, #67300, #58183 ) ;
#95569=DIRECTION ( 'NONE',  ( 0.000000000000000000, -0.9999939076577903929, 0.003490651415223739937 ) ) ;
#95570=CIRCLE ( 'NONE', #28675, 0.06509327318403745899 ) ;
#95571=CARTESIAN_POINT ( 'NONE',  ( 14.19999999999989626, 12.50000000000000000, -0.06509327318403970719 ) ) ;
#95572=EDGE_CURVE ( 'NONE', #46914, #103864, #63690, .T. ) ;
#95573=CARTESIAN_POINT ( 'NONE',  ( 0.8499999999999527933, 12.50000000000000000, 7.188010851410848723 ) ) ;
#95574=VERTEX_POINT ( 'NONE', #64319 ) ;
#95575=DIRECTION ( 'NONE',  ( 0.000000000000000000, -0.000000000000000000, 1.000000000000000000 ) ) ;
#95576=ADVANCED_FACE ( 'NONE', ( #14562 ), #99271, .T. ) ;
#95577=VECTOR ( 'NONE', #58096, 1000.000000000000000 ) ;
#95578=AXIS2_PLACEMENT_3D ( 'NONE', #23032, #20880, #68682 ) ;
#95579=DIRECTION ( 'NONE',  ( -4.274815082592931898E-19, -0.9999939076577903929, -0.003490651415223739937 ) ) ;
#95580=ORIENTED_EDGE ( 'NONE', *, *, #125098, .F. ) ;
#95581=EDGE_LOOP ( 'NONE', ( #35971, #76150 ) ) ;
#95582=ORIENTED_EDGE ( 'NONE', *, *, #14063, .T. ) ;
#95583=DIRECTION ( 'NONE',  ( 0.000000000000000000, 0.000000000000000000, 1.000000000000000000 ) ) ;
#95584=AXIS2_PLACEMENT_3D ( 'NONE', #82213, #31822, #80931 ) ;
#95585=AXIS2_PLACEMENT_3D ( 'NONE', #55544, #45726, #102690 ) ;
#95586=DIRECTION ( 'NONE',  ( -0.000000000000000000, -1.000000000000000000, -0.000000000000000000 ) ) ;
#95588=EDGE_LOOP ( 'NONE', ( #11953, #101759, #30481, #68455 ) ) ;
#95589=DIRECTION ( 'NONE',  ( -0.000000000000000000, -1.000000000000000000, -0.000000000000000000 ) ) ;
#95590=CARTESIAN_POINT ( 'NONE',  ( 6.249999999999965361, 2.500000000000000000, 2.065063509461097624 ) ) ;
#95591=FACE_OUTER_BOUND ( 'NONE', #55593, .T. ) ;
#95592=CARTESIAN_POINT ( 'NONE',  ( -11.64999999999999680, 2.500000000000000000, 5.802370205355744659 ) ) ;
#95593=EDGE_CURVE ( 'NONE', #70324, #13448, #53210, .T. ) ;
#95594=DIRECTION ( 'NONE',  ( 0.000000000000000000, 0.000000000000000000, 1.000000000000000000 ) ) ;
#95595=ORIENTED_EDGE ( 'NONE', *, *, #14852, .T. ) ;
#95596=CONICAL_SURFACE ( 'NONE', #106057, 0.09999999999999999167, 0.003490658503988666988 ) ;
#95597=DIRECTION ( 'NONE',  ( 0.000000000000000000, 1.000000000000000000, 0.000000000000000000 ) ) ;
#95598=ORIENTED_EDGE ( 'NONE', *, *, #124478, .T. ) ;
#95599=ORIENTED_EDGE ( 'NONE', *, *, #71898, .F. ) ;
#95600=ORIENTED_EDGE ( 'NONE', *, *, #96237, .F. ) ;
#95601=LINE ( 'NONE', #15066, #33553 ) ;
#95602=FACE_BOUND ( 'NONE', #97353, .T. ) ;
#95603=CARTESIAN_POINT ( 'NONE',  ( 8.099999999999921485, 2.500000000000000000, 0.3464101615137735735 ) ) ;
#95604=CIRCLE ( 'NONE', #62171, 0.1000000000000000472 ) ;
#95605=DIRECTION ( 'NONE',  ( -0.000000000000000000, -1.000000000000000000, -0.000000000000000000 ) ) ;
#95607=EDGE_CURVE ( 'NONE', #40320, #14309, #75420, .T. ) ;
#95609=DIRECTION ( 'NONE',  ( 0.000000000000000000, 0.000000000000000000, 1.000000000000000000 ) ) ;
#95610=DIRECTION ( 'NONE',  ( -4.274815082592931898E-19, -0.9999939076577903929, -0.003490651415223739937 ) ) ;
#95611=VECTOR ( 'NONE', #92594, 1000.000000000000000 ) ;
#95612=DIRECTION ( 'NONE',  ( 0.000000000000000000, -0.000000000000000000, 1.000000000000000000 ) ) ;
#95613=AXIS2_PLACEMENT_3D ( 'NONE', #95326, #125430, #26589 ) ;
#95614=PLANE ( 'NONE',  #122080 ) ;
#95615=EDGE_LOOP ( 'NONE', ( #123292, #104558, #121143, #4053 ) ) ;
#95616=LINE ( 'NONE', #6542, #122192 ) ;
#95617=AXIS2_PLACEMENT_3D ( 'NONE', #30368, #21164, #91203 ) ;
#95618=VECTOR ( 'NONE', #126343, 1000.000000000000000 ) ;
#95619=DIRECTION ( 'NONE',  ( -0.000000000000000000, 1.000000000000000000, -0.000000000000000000 ) ) ;
#95620=ORIENTED_EDGE ( 'NONE', *, *, #6548, .F. ) ;
#95621=DIRECTION ( 'NONE',  ( 0.000000000000000000, 1.000000000000000000, 0.000000000000000000 ) ) ;
#95622=CIRCLE ( 'NONE', #68424, 0.06509327318403745899 ) ;
#95623=EDGE_CURVE ( 'NONE', #100019, #113079, #90844, .T. ) ;
#95624=FACE_BOUND ( 'NONE', #2392, .T. ) ;
#95626=AXIS2_PLACEMENT_3D ( 'NONE', #57872, #29065, #29693 ) ;
#95627=CIRCLE ( 'NONE', #103948, 0.06509327318403745899 ) ;
#95628=EDGE_LOOP ( 'NONE', ( #97568, #667 ) ) ;
#95629=CARTESIAN_POINT ( 'NONE',  ( 7.099999999999928590, 12.50000000000000000, -4.395220292106239768 ) ) ;
#95630=CARTESIAN_POINT ( 'NONE',  ( 3.749999999999975131, 2.500000000000000000, 6.395190528383296602 ) ) ;
#95631=ORIENTED_EDGE ( 'NONE', *, *, #26797, .T. ) ;
#95632=EDGE_LOOP ( 'NONE', ( #48049, #37653 ) ) ;
#95634=ORIENTED_EDGE ( 'NONE', *, *, #3758, .F. ) ;
#95636=CARTESIAN_POINT ( 'NONE',  ( -1.850000000000033396, 12.50000000000000000, -2.576566944158915184 ) ) ;
#95637=CARTESIAN_POINT ( 'NONE',  ( -3.350000000000028511, 2.500000000000000000, 1.372243186433545370 ) ) ;
#95638=CARTESIAN_POINT ( 'NONE',  ( -4.400000000000025224, 12.50000000000000000, -0.2813168883297409439 ) ) ;
#95639=CARTESIAN_POINT ( 'NONE',  ( -1.250000000000037970, 12.50000000000000000, 2.792790559304612064 ) ) ;
#95640=CONICAL_SURFACE ( 'NONE', #53777, 0.09999999999999999167, 0.003490658503988666988 ) ;
#95641=VERTEX_POINT ( 'NONE', #104249 ) ;
#95642=EDGE_CURVE ( 'NONE', #30305, #35899, #86639, .T. ) ;
#95643=ORIENTED_EDGE ( 'NONE', *, *, #32308, .F. ) ;
#95644=DIRECTION ( 'NONE',  ( 0.000000000000000000, 0.000000000000000000, 1.000000000000000000 ) ) ;
#95646=DIRECTION ( 'NONE',  ( -0.000000000000000000, 1.000000000000000000, -0.000000000000000000 ) ) ;
#95647=CARTESIAN_POINT ( 'NONE',  ( 10.39999999999991331, 2.500000000000000000, -2.385244779468109755E-15 ) ) ;
#95648=EDGE_LOOP ( 'NONE', ( #124982, #103276, #92973, #60616 ) ) ;
#95649=ORIENTED_EDGE ( 'NONE', *, *, #109226, .F. ) ;
#95650=DIRECTION ( 'NONE',  ( 0.000000000000000000, 0.000000000000000000, 1.000000000000000000 ) ) ;
#95651=ORIENTED_EDGE ( 'NONE', *, *, #20867, .F. ) ;
#95652=PLANE ( 'NONE',  #124502 ) ;
#95653=CARTESIAN_POINT ( 'NONE',  ( -10.00000000000000533, 12.50000000000000000, 0.6277270498435120194 ) ) ;
#95654=ORIENTED_EDGE ( 'NONE', *, *, #92568, .T. ) ;
#95655=DIRECTION ( 'NONE',  ( 0.000000000000000000, -0.000000000000000000, 1.000000000000000000 ) ) ;
#95656=EDGE_CURVE ( 'NONE', #42231, #18847, #114071, .T. ) ;
#95657=DIRECTION ( 'NONE',  ( 0.000000000000000000, 0.000000000000000000, 1.000000000000000000 ) ) ;
#95658=AXIS2_PLACEMENT_3D ( 'NONE', #48681, #68303, #87297 ) ;
#95659=DIRECTION ( 'NONE',  ( 0.000000000000000000, 1.000000000000000000, 0.000000000000000000 ) ) ;
#95660=FACE_OUTER_BOUND ( 'NONE', #89325, .T. ) ;
#95661=CARTESIAN_POINT ( 'NONE',  ( 11.04999999999990656, 2.500000000000000000, 2.511473670974873507 ) ) ;
#95662=DIRECTION ( 'NONE',  ( -4.274815082592931898E-19, -0.9999939076577903929, -0.003490651415223739937 ) ) ;
#95663=EDGE_CURVE ( 'NONE', #97017, #40454, #76184, .T. ) ;
#95664=EDGE_CURVE ( 'NONE', #76810, #66380, #35521, .T. ) ;
#95665=DIRECTION ( 'NONE',  ( 0.000000000000000000, 0.000000000000000000, 1.000000000000000000 ) ) ;
#95667=ADVANCED_FACE ( 'NONE', ( #103614 ), #85252, .T. ) ;
#95668=EDGE_CURVE ( 'NONE', #54565, #81006, #104872, .T. ) ;
#95669=CARTESIAN_POINT ( 'NONE',  ( 3.099999999999945466, 2.500000000000000000, -3.983716857408426293 ) ) ;
#95670=AXIS2_PLACEMENT_3D ( 'NONE', #69176, #60681, #98002 ) ;
#95671=ORIENTED_EDGE ( 'NONE', *, *, #71147, .F. ) ;
#95672=AXIS2_PLACEMENT_3D ( 'NONE', #34852, #25642, #123837 ) ;
#95673=CIRCLE ( 'NONE', #39266, 0.06509327318403745899 ) ;
#95674=ORIENTED_EDGE ( 'NONE', *, *, #37165, .F. ) ;
#95675=CARTESIAN_POINT ( 'NONE',  ( 2.049999999999950084, 12.50000000000000000, 2.230156782645134950 ) ) ;
#95676=VERTEX_POINT ( 'NONE', #115323 ) ;
#95677=ADVANCED_FACE ( 'NONE', ( #36163 ), #46952, .T. ) ;
#95678=CARTESIAN_POINT ( 'NONE',  ( 4.599999999999937472, 2.500000000000000000, 0.6928203230275494784 ) ) ;
#95679=EDGE_CURVE ( 'NONE', #42325, #89946, #25679, .T. ) ;
#95680=EDGE_LOOP ( 'NONE', ( #123920, #41813 ) ) ;
#95681=VERTEX_POINT ( 'NONE', #4732 ) ;
#95682=ORIENTED_EDGE ( 'NONE', *, *, #51381, .T. ) ;
#95683=EDGE_CURVE ( 'NONE', #52044, #95641, #88792, .T. ) ;
#95684=DIRECTION ( 'NONE',  ( -0.000000000000000000, -1.000000000000000000, -0.000000000000000000 ) ) ;
#95685=EDGE_CURVE ( 'NONE', #23954, #95574, #26342, .T. ) ;
#95686=AXIS2_PLACEMENT_3D ( 'NONE', #15121, #53153, #55077 ) ;
#95687=ADVANCED_FACE ( 'NONE', ( #74796 ), #114702, .T. ) ;
#95688=CARTESIAN_POINT ( 'NONE',  ( 12.29999999999990656, 12.50000000000000000, 3.918623584224383727 ) ) ;
#95690=CARTESIAN_POINT ( 'NONE',  ( 2.899999999999946620, 12.50000000000000000, -0.6928203230275542523 ) ) ;
#95691=CARTESIAN_POINT ( 'NONE',  ( 6.449999999999930012, 12.50000000000000000, 1.753560074763284016 ) ) ;
#95692=LINE ( 'NONE', #84576, #114439 ) ;
#95693=CIRCLE ( 'NONE', #83262, 0.1000000000000002554 ) ;
#95694=ORIENTED_EDGE ( 'NONE', *, *, #77988, .T. ) ;
#95695=EDGE_CURVE ( 'NONE', #98508, #6453, #63672, .T. ) ;
#95696=CARTESIAN_POINT ( 'NONE',  ( 8.749999999999923617, 2.500000000000000000, -7.088010851410853519 ) ) ;
#95697=ORIENTED_EDGE ( 'NONE', *, *, #92894, .T. ) ;
#95698=VERTEX_POINT ( 'NONE', #96427 ) ;
#95699=ORIENTED_EDGE ( 'NONE', *, *, #61518, .T. ) ;
#95700=ORIENTED_EDGE ( 'NONE', *, *, #68764, .F. ) ;
#95701=DIRECTION ( 'NONE',  ( 0.000000000000000000, -0.000000000000000000, 1.000000000000000000 ) ) ;
#95702=ORIENTED_EDGE ( 'NONE', *, *, #78736, .T. ) ;
#95704=CIRCLE ( 'NONE', #122790, 0.1000000000000000472 ) ;
#95705=CONICAL_SURFACE ( 'NONE', #39299, 0.09999999999999982514, 0.003490658503988666988 ) ;
#95706=CARTESIAN_POINT ( 'NONE',  ( -6.650000000000014566, 2.500000000000000000, 5.702370205355745014 ) ) ;
#95707=FACE_OUTER_BOUND ( 'NONE', #74659, .T. ) ;
#95708=CARTESIAN_POINT ( 'NONE',  ( 0.3999999999999628852, 12.50000000000000000, -0.6928203230275520319 ) ) ;
#95709=AXIS2_PLACEMENT_3D ( 'NONE', #55187, #95112, #113456 ) ;
#95710=DIRECTION ( 'NONE',  ( 0.000000000000000000, -0.000000000000000000, 1.000000000000000000 ) ) ;
#95711=DIRECTION ( 'NONE',  ( 0.000000000000000000, -0.000000000000000000, 1.000000000000000000 ) ) ;
#95712=CARTESIAN_POINT ( 'NONE',  ( 2.299999999999948752, 2.500000000000000000, 0.3464101615137735735 ) ) ;
#95713=ORIENTED_EDGE ( 'NONE', *, *, #66214, .F. ) ;
#95714=DIRECTION ( 'NONE',  ( 0.000000000000000000, 1.000000000000000000, 0.000000000000000000 ) ) ;
#95715=AXIS2_PLACEMENT_3D ( 'NONE', #48161, #18038, #28523 ) ;
#95716=ORIENTED_EDGE ( 'NONE', *, *, #115899, .F. ) ;
#95717=DIRECTION ( 'NONE',  ( 0.000000000000000000, 0.000000000000000000, 1.000000000000000000 ) ) ;
#95718=ORIENTED_EDGE ( 'NONE', *, *, #12039, .F. ) ;
#95719=DIRECTION ( 'NONE',  ( -4.274815082592931898E-19, -0.9999939076577903929, -0.003490651415223739937 ) ) ;
#95720=ORIENTED_EDGE ( 'NONE', *, *, #88836, .T. ) ;
#95721=AXIS2_PLACEMENT_3D ( 'NONE', #29217, #129361, #118866 ) ;
#95722=EDGE_LOOP ( 'NONE', ( #126556, #43020, #100678, #19594 ) ) ;
#95723=CARTESIAN_POINT ( 'NONE',  ( 3.749999999999944045, 2.500000000000000000, -2.957883832488653830 ) ) ;
#95724=CARTESIAN_POINT ( 'NONE',  ( -13.09999999999999254, 2.500000000000000000, -3.983716857408423628 ) ) ;
#95725=EDGE_CURVE ( 'NONE', #58662, #53518, #48003, .T. ) ;
#95726=CIRCLE ( 'NONE', #51816, 0.06509327318403745899 ) ;
#95727=AXIS2_PLACEMENT_3D ( 'NONE', #67564, #78046, #57112 ) ;
#95728=FACE_OUTER_BOUND ( 'NONE', #35044, .T. ) ;
#95729=DIRECTION ( 'NONE',  ( 0.000000000000000000, 0.000000000000000000, -1.000000000000000000 ) ) ;
#95730=EDGE_CURVE ( 'NONE', #53628, #53022, #26103, .T. ) ;
#95731=DIRECTION ( 'NONE',  ( 0.000000000000000000, 0.000000000000000000, 1.000000000000000000 ) ) ;
#95732=ORIENTED_EDGE ( 'NONE', *, *, #59205, .T. ) ;
#95733=DIRECTION ( 'NONE',  ( 0.000000000000000000, 0.000000000000000000, 1.000000000000000000 ) ) ;
#95734=LINE ( 'NONE', #97654, #20095 ) ;
#95735=CARTESIAN_POINT ( 'NONE',  ( 0.8499999999999553468, 12.50000000000000000, -2.857883832488653741 ) ) ;
#95736=DIRECTION ( 'NONE',  ( -4.274815082592931898E-19, -0.9999939076577903929, -0.003490651415223739937 ) ) ;
#95737=ADVANCED_FACE ( 'NONE', ( #17202 ), #99171, .T. ) ;
#95738=FACE_OUTER_BOUND ( 'NONE', #36220, .T. ) ;
#95739=EDGE_LOOP ( 'NONE', ( #9024, #12866, #91143, #87298 ) ) ;
#95740=VERTEX_POINT ( 'NONE', #6738 ) ;
#95741=ORIENTED_EDGE ( 'NONE', *, *, #75159, .F. ) ;
#95742=FACE_OUTER_BOUND ( 'NONE', #119032, .T. ) ;
#95743=CARTESIAN_POINT ( 'NONE',  ( -9.550000000000006040, 12.50000000000000000, -2.165063509461101710 ) ) ;
#95744=CIRCLE ( 'NONE', #76964, 0.1000000000000000056 ) ;
#95746=CARTESIAN_POINT ( 'NONE',  ( -8.950000000000009948, 2.500000000000000000, 2.611473670974873151 ) ) ;
#95747=LINE ( 'NONE', #104900, #13101 ) ;
#95748=DIRECTION ( 'NONE',  ( -0.000000000000000000, -1.000000000000000000, -0.000000000000000000 ) ) ;
#95749=DIRECTION ( 'NONE',  ( 0.000000000000000000, 0.000000000000000000, 1.000000000000000000 ) ) ;
#95750=ORIENTED_EDGE ( 'NONE', *, *, #46331, .T. ) ;
#95751=AXIS2_PLACEMENT_3D ( 'NONE', #49191, #107438, #108720 ) ;
#95752=VECTOR ( 'NONE', #122484, 1000.000000000000000 ) ;
#95753=CARTESIAN_POINT ( 'NONE',  ( -14.99999999999998401, 2.500000000000000000, 0.5928203230275517210 ) ) ;
#95754=CARTESIAN_POINT ( 'NONE',  ( -8.950000000000009948, 12.50000000000000000, 2.511473670974873507 ) ) ;
#95755=ORIENTED_EDGE ( 'NONE', *, *, #122695, .T. ) ;
#95756=DIRECTION ( 'NONE',  ( 0.000000000000000000, 1.000000000000000000, 0.000000000000000000 ) ) ;
#95757=FACE_OUTER_BOUND ( 'NONE', #70490, .T. ) ;
#95758=CIRCLE ( 'NONE', #18387, 0.06509327318403745899 ) ;
#95759=CARTESIAN_POINT ( 'NONE',  ( -10.00000000000000355, 2.500000000000000000, -0.7928203230275542301 ) ) ;
#95760=AXIS2_PLACEMENT_3D ( 'NONE', #117789, #99480, #48430 ) ;
#95761=ORIENTED_EDGE ( 'NONE', *, *, #87938, .F. ) ;
#95762=DIRECTION ( 'NONE',  ( -0.000000000000000000, 1.000000000000000000, -0.000000000000000000 ) ) ;
#95763=ORIENTED_EDGE ( 'NONE', *, *, #34707, .F. ) ;
#95764=LINE ( 'NONE', #105593, #2030 ) ;
#95765=CARTESIAN_POINT ( 'NONE',  ( -13.14999999999999147, 12.50000000000000000, 1.753560074763288013 ) ) ;
#95766=EDGE_LOOP ( 'NONE', ( #33785, #9911, #83217, #14994 ) ) ;
#95767=DIRECTION ( 'NONE',  ( -0.000000000000000000, -1.000000000000000000, -0.000000000000000000 ) ) ;
#95768=DIRECTION ( 'NONE',  ( 0.000000000000000000, -0.000000000000000000, 1.000000000000000000 ) ) ;
#95769=EDGE_CURVE ( 'NONE', #100605, #93533, #42853, .T. ) ;
#95770=AXIS2_PLACEMENT_3D ( 'NONE', #91216, #82701, #1533 ) ;
#95771=ORIENTED_EDGE ( 'NONE', *, *, #70567, .T. ) ;
#95772=EDGE_CURVE ( 'NONE', #129184, #83779, #42764, .T. ) ;
#95773=ORIENTED_EDGE ( 'NONE', *, *, #94034, .T. ) ;
#95774=CARTESIAN_POINT ( 'NONE',  ( 5.599999999999934808, 2.500000000000000000, -3.983716857408426293 ) ) ;
#95775=AXIS2_PLACEMENT_3D ( 'NONE', #74471, #84928, #105210 ) ;
#95776=ORIENTED_EDGE ( 'NONE', *, *, #49902, .F. ) ;
#95777=AXIS2_PLACEMENT_3D ( 'NONE', #69591, #47386, #49338 ) ;
#95778=DIRECTION ( 'NONE',  ( 0.000000000000000000, 0.000000000000000000, 1.000000000000000000 ) ) ;
#95779=DIRECTION ( 'NONE',  ( 0.000000000000000000, 0.000000000000000000, -1.000000000000000000 ) ) ;
#95780=EDGE_CURVE ( 'NONE', #6261, #39515, #115882, .T. ) ;
#95781=ORIENTED_EDGE ( 'NONE', *, *, #2863, .F. ) ;
#95782=CONICAL_SURFACE ( 'NONE', #26737, 0.09999999999999982514, 0.003490658503988666988 ) ;
#95783=FACE_OUTER_BOUND ( 'NONE', #52698, .T. ) ;
#95784=DIRECTION ( 'NONE',  ( 0.000000000000000000, -0.000000000000000000, 1.000000000000000000 ) ) ;
#95785=VECTOR ( 'NONE', #10815, 1000.000000000000000 ) ;
#95786=VERTEX_POINT ( 'NONE', #87892 ) ;
#95787=FACE_OUTER_BOUND ( 'NONE', #116657, .T. ) ;
#95788=CARTESIAN_POINT ( 'NONE',  ( -4.400000000000025224, 2.500000000000000000, 4.676537180435972552 ) ) ;
#95789=AXIS2_PLACEMENT_3D ( 'NONE', #68859, #108777, #29582 ) ;
#95790=DIRECTION ( 'NONE',  ( -0.000000000000000000, 1.000000000000000000, -0.000000000000000000 ) ) ;
#95791=PLANE ( 'NONE',  #13193 ) ;
#95792=DIRECTION ( 'NONE',  ( 0.000000000000000000, -0.000000000000000000, 1.000000000000000000 ) ) ;
#95793=AXIS2_PLACEMENT_3D ( 'NONE', #96939, #84552, #27541 ) ;
#95794=DIRECTION ( 'NONE',  ( 0.000000000000000000, 0.000000000000000000, 1.000000000000000000 ) ) ;
#95795=EDGE_LOOP ( 'NONE', ( #100040, #54941 ) ) ;
#95796=ORIENTED_EDGE ( 'NONE', *, *, #96084, .T. ) ;
#95797=ORIENTED_EDGE ( 'NONE', *, *, #30403, .T. ) ;
#95798=ORIENTED_EDGE ( 'NONE', *, *, #82567, .F. ) ;
#95799=CARTESIAN_POINT ( 'NONE',  ( 32.25969448929755856, 3.190781364619325267, 3.146220011503479075 ) ) ;
#95801=CARTESIAN_POINT ( 'NONE',  ( 8.349999999999923261, 2.500000000000000000, 2.165063509461097713 ) ) ;
#95802=VERTEX_POINT ( 'NONE', #127836 ) ;
#95803=FACE_BOUND ( 'NONE', #12012, .T. ) ;
#95804=FACE_OUTER_BOUND ( 'NONE', #103431, .T. ) ;
#95805=DIRECTION ( 'NONE',  ( 0.000000000000000000, 0.000000000000000000, 1.000000000000000000 ) ) ;
#95806=CARTESIAN_POINT ( 'NONE',  ( 10.19999999999991402, 12.50000000000000000, 0.3464101615137735735 ) ) ;
#95807=EDGE_CURVE ( 'NONE', #40951, #34456, #19846, .T. ) ;
#95808=CIRCLE ( 'NONE', #39404, 0.09999999999999982514 ) ;
#95809=CIRCLE ( 'NONE', #72834, 0.06509327318403745899 ) ;
#95810=DIRECTION ( 'NONE',  ( 0.000000000000000000, 0.000000000000000000, -1.000000000000000000 ) ) ;
#95811=DIRECTION ( 'NONE',  ( 0.000000000000000000, 0.000000000000000000, -1.000000000000000000 ) ) ;
#95812=DIRECTION ( 'NONE',  ( 0.000000000000000000, -0.9999939076577903929, 0.003490651415223739937 ) ) ;
#95813=DIRECTION ( 'NONE',  ( -0.000000000000000000, 1.000000000000000000, -0.000000000000000000 ) ) ;
#95814=DIRECTION ( 'NONE',  ( 0.000000000000000000, 0.000000000000000000, 1.000000000000000000 ) ) ;
#95815=EDGE_CURVE ( 'NONE', #55120, #99646, #9463, .T. ) ;
#95816=EDGE_CURVE ( 'NONE', #4150, #46427, #105614, .T. ) ;
#95817=DIRECTION ( 'NONE',  ( -0.000000000000000000, 1.000000000000000000, -0.000000000000000000 ) ) ;
#95818=EDGE_CURVE ( 'NONE', #117477, #96527, #82637, .T. ) ;
#95819=ADVANCED_FACE ( 'NONE', ( #116718 ), #30322, .T. ) ;
#95820=DIRECTION ( 'NONE',  ( -0.000000000000000000, -1.000000000000000000, -0.000000000000000000 ) ) ;
#95821=ORIENTED_EDGE ( 'NONE', *, *, #120822, .F. ) ;
#95822=VERTEX_POINT ( 'NONE', #55868 ) ;
#95823=EDGE_LOOP ( 'NONE', ( #18025, #25098 ) ) ;
#95824=VERTEX_POINT ( 'NONE', #85960 ) ;
#95825=DIRECTION ( 'NONE',  ( 0.000000000000000000, 0.000000000000000000, 1.000000000000000000 ) ) ;
#95826=ADVANCED_FACE ( 'NONE', ( #7403 ), #78442, .T. ) ;
#95827=VERTEX_POINT ( 'NONE', #46704 ) ;
#95828=AXIS2_PLACEMENT_3D ( 'NONE', #20449, #99660, #11907 ) ;
#95829=CARTESIAN_POINT ( 'NONE',  ( 16.56576425165006583, 1.500000000000000888, -6.084390597445814564 ) ) ;
#95830=EDGE_CURVE ( 'NONE', #112983, #6303, #45425, .T. ) ;
#95831=VERTEX_POINT ( 'NONE', #86618 ) ;
#95832=ORIENTED_EDGE ( 'NONE', *, *, #5116, .F. ) ;
#95833=DIRECTION ( 'NONE',  ( 0.000000000000000000, 0.000000000000000000, 1.000000000000000000 ) ) ;
#95834=CIRCLE ( 'NONE', #79404, 0.06509327318403745899 ) ;
#95836=CONICAL_SURFACE ( 'NONE', #91909, 0.09999999999999982514, 0.003490658503988666988 ) ;
#95837=CARTESIAN_POINT ( 'NONE',  ( 10.89704209861766770, -2.500000000000253131, 8.980393935570946340 ) ) ;
#95838=CIRCLE ( 'NONE', #127241, 0.06509327318403745899 ) ;
#95839=CARTESIAN_POINT ( 'NONE',  ( 4.349999999999937472, 12.50000000000000000, 6.906693963081109722 ) ) ;
#95840=DIRECTION ( 'NONE',  ( 0.000000000000000000, -0.000000000000000000, 1.000000000000000000 ) ) ;
#95841=DIRECTION ( 'NONE',  ( -0.000000000000000000, 1.000000000000000000, -0.000000000000000000 ) ) ;
#95842=EDGE_CURVE ( 'NONE', #2195, #51573, #125887, .T. ) ;
#95843=ORIENTED_EDGE ( 'NONE', *, *, #76457, .T. ) ;
#95845=AXIS2_PLACEMENT_3D ( 'NONE', #25627, #6604, #127078 ) ;
#95846=AXIS2_PLACEMENT_3D ( 'NONE', #30836, #91664, #92302 ) ;
#95847=ORIENTED_EDGE ( 'NONE', *, *, #5892, .F. ) ;
#95848=VECTOR ( 'NONE', #31317, 1000.000000000000000 ) ;
#95849=ORIENTED_EDGE ( 'NONE', *, *, #11406, .T. ) ;
#95850=ORIENTED_EDGE ( 'NONE', *, *, #71143, .F. ) ;
#95851=PLANE ( 'NONE',  #63002 ) ;
#95852=ORIENTED_EDGE ( 'NONE', *, *, #26333, .T. ) ;
#95853=EDGE_LOOP ( 'NONE', ( #67027, #37582 ) ) ;
#95854=AXIS2_PLACEMENT_3D ( 'NONE', #48937, #48282, #107188 ) ;
#95855=FACE_OUTER_BOUND ( 'NONE', #84113, .T. ) ;
#95856=CIRCLE ( 'NONE', #56127, 0.1000000000000002554 ) ;
#95857=CARTESIAN_POINT ( 'NONE',  ( -3.100000000000028511, 2.500000000000000000, -0.2464101615137782308 ) ) ;
#95858=DIRECTION ( 'NONE',  ( 0.000000000000000000, -0.9999939076577903929, 0.003490651415223739937 ) ) ;
#95860=FACE_OUTER_BOUND ( 'NONE', #72767, .T. ) ;
#95861=CARTESIAN_POINT ( 'NONE',  ( 0.8499999999999553468, 2.500000000000000000, 2.265063509461097357 ) ) ;
#95862=ORIENTED_EDGE ( 'NONE', *, *, #88459, .T. ) ;
#95863=DIRECTION ( 'NONE',  ( 0.000000000000000000, 1.000000000000000000, 0.000000000000000000 ) ) ;
#95864=AXIS2_PLACEMENT_3D ( 'NONE', #55892, #95185, #55264 ) ;
#95865=ORIENTED_EDGE ( 'NONE', *, *, #8946, .T. ) ;
#95866=DIRECTION ( 'NONE',  ( 0.000000000000000000, 0.000000000000000000, 1.000000000000000000 ) ) ;
#95867=ORIENTED_EDGE ( 'NONE', *, *, #19772, .T. ) ;
#95868=CARTESIAN_POINT ( 'NONE',  ( 10.19999999999991047, 2.500000000000000000, -3.983716857408426293 ) ) ;
#95869=DIRECTION ( 'NONE',  ( 0.000000000000000000, 0.000000000000000000, 1.000000000000000000 ) ) ;
#95870=CONICAL_SURFACE ( 'NONE', #28976, 0.1000000000000002554, 0.003490658503988666988 ) ;
#95871=AXIS2_PLACEMENT_3D ( 'NONE', #79944, #40035, #22335 ) ;
#95872=EDGE_LOOP ( 'NONE', ( #127769, #40947 ) ) ;
#95873=CARTESIAN_POINT ( 'NONE',  ( -10.85000000000000142, 12.50000000000000000, -1.472243186433546125 ) ) ;
#95874=CARTESIAN_POINT ( 'NONE',  ( 1.049999999999952971, 12.50000000000000000, 6.083687093685483660 ) ) ;
#95875=EDGE_LOOP ( 'NONE', ( #112682, #94023 ) ) ;
#95876=FILL_AREA_STYLE ('',( #34397 ) ) ;
#95877=EDGE_CURVE ( 'NONE', #29719, #10941, #53299, .T. ) ;
#95879=CARTESIAN_POINT ( 'NONE',  ( 4.549999999999939426, 2.500000000000000000, -2.165063509461101710 ) ) ;
#95880=EDGE_CURVE ( 'NONE', #64833, #124839, #26192, .T. ) ;
#95881=ORIENTED_EDGE ( 'NONE', *, *, #54810, .F. ) ;
#95882=ORIENTED_EDGE ( 'NONE', *, *, #48531, .F. ) ;
#95884=CARTESIAN_POINT ( 'NONE',  ( 97.50000000000000000, 0.000000000000000000, 0.000000000000000000 ) ) ;
#95886=DIRECTION ( 'NONE',  ( -0.000000000000000000, -1.000000000000000000, -0.000000000000000000 ) ) ;
#95887=AXIS2_PLACEMENT_3D ( 'NONE', #39697, #31155, #111631 ) ;
#95888=VECTOR ( 'NONE', #59572, 1000.000000000000000 ) ;
#95889=DIRECTION ( 'NONE',  ( -0.000000000000000000, -1.000000000000000000, -0.000000000000000000 ) ) ;
#95890=DIRECTION ( 'NONE',  ( 0.000000000000000000, 0.000000000000000000, 1.000000000000000000 ) ) ;
#95892=ORIENTED_EDGE ( 'NONE', *, *, #122340, .T. ) ;
#95893=LINE ( 'NONE', #115507, #31830 ) ;
#95894=ORIENTED_EDGE ( 'NONE', *, *, #24897, .F. ) ;
#95895=AXIS2_PLACEMENT_3D ( 'NONE', #124423, #95605, #43298 ) ;
#95896=AXIS2_PLACEMENT_3D ( 'NONE', #42362, #71163, #80989 ) ;
#95897=CARTESIAN_POINT ( 'NONE',  ( -10.45000000000000462, 2.500000000000000000, -2.165063509461097713 ) ) ;
#95898=CARTESIAN_POINT ( 'NONE',  ( -0.6500000000000403233, 2.500000000000000000, 6.248780366869520542 ) ) ;
#95899=DIRECTION ( 'NONE',  ( 0.000000000000000000, 1.000000000000000000, 0.000000000000000000 ) ) ;
#95900=ORIENTED_EDGE ( 'NONE', *, *, #1792, .T. ) ;
#95901=AXIS2_PLACEMENT_3D ( 'NONE', #54570, #4824, #84689 ) ;
#95902=CARTESIAN_POINT ( 'NONE',  ( 3.099999999999945466, 2.500000000000000000, 0.3464101615137735735 ) ) ;
#95903=DIRECTION ( 'NONE',  ( -0.000000000000000000, -1.000000000000000000, -0.000000000000000000 ) ) ;
#95904=ORIENTED_EDGE ( 'NONE', *, *, #29468, .T. ) ;
#95905=CARTESIAN_POINT ( 'NONE',  ( -11.24999999999999822, 12.50000000000000000, 1.537336459617582918 ) ) ;
#95906=EDGE_CURVE ( 'NONE', #87583, #23954, #95145, .T. ) ;
#95907=VERTEX_POINT ( 'NONE', #61026 ) ;
#95908=ORIENTED_EDGE ( 'NONE', *, *, #21344, .T. ) ;
#95910=AXIS2_PLACEMENT_3D ( 'NONE', #84366, #35285, #63443 ) ;
#95911=ORIENTED_EDGE ( 'NONE', *, *, #115264, .F. ) ;
#95912=DIRECTION ( 'NONE',  ( 0.000000000000000000, 1.000000000000000000, 0.000000000000000000 ) ) ;
#95914=DIRECTION ( 'NONE',  ( 0.000000000000000000, -0.000000000000000000, 1.000000000000000000 ) ) ;
#95915=EDGE_CURVE ( 'NONE', #29584, #32403, #86727, .T. ) ;
#95916=ORIENTED_EDGE ( 'NONE', *, *, #77026, .F. ) ;
#95917=CONICAL_SURFACE ( 'NONE', #64516, 0.1000000000000002554, 0.003490658503988666988 ) ;
#95918=FACE_BOUND ( 'NONE', #31571, .T. ) ;
#95919=AXIS2_PLACEMENT_3D ( 'NONE', #31026, #108892, #30372 ) ;
#95920=FACE_OUTER_BOUND ( 'NONE', #54223, .T. ) ;
#95921=ORIENTED_EDGE ( 'NONE', *, *, #54881, .T. ) ;
#95922=EDGE_CURVE ( 'NONE', #112250, #84669, #103464, .T. ) ;
#95923=CARTESIAN_POINT ( 'NONE',  ( 3.949999999999942446, 12.50000000000000000, -6.841600689897078702 ) ) ;
#95924=FACE_OUTER_BOUND ( 'NONE', #101821, .T. ) ;
#95925=EDGE_CURVE ( 'NONE', #29739, #118702, #124396, .T. ) ;
#95926=AXIS2_PLACEMENT_3D ( 'NONE', #35683, #106348, #48084 ) ;
#95927=VERTEX_POINT ( 'NONE', #49949 ) ;
#95928=AXIS2_PLACEMENT_3D ( 'NONE', #46422, #48363, #7132 ) ;
#95929=AXIS2_PLACEMENT_3D ( 'NONE', #18738, #58675, #8904 ) ;
#95930=ORIENTED_EDGE ( 'NONE', *, *, #50141, .F. ) ;
#95931=VERTEX_POINT ( 'NONE', #39489 ) ;
#95932=DIRECTION ( 'NONE',  ( 0.000000000000000000, 1.000000000000000000, 0.000000000000000000 ) ) ;
#95933=DIRECTION ( 'NONE',  ( 0.000000000000000000, -0.000000000000000000, 1.000000000000000000 ) ) ;
#95934=DIRECTION ( 'NONE',  ( 0.000000000000000000, 1.000000000000000000, 0.000000000000000000 ) ) ;
#95935=EDGE_CURVE ( 'NONE', #117161, #98934, #22008, .T. ) ;
#95936=FACE_BOUND ( 'NONE', #59741, .T. ) ;
#95937=VERTEX_POINT ( 'NONE', #118654 ) ;
#95939=CONICAL_SURFACE ( 'NONE', #8105, 0.1000000000000002554, 0.003490658503988666988 ) ;
#95940=DIRECTION ( 'NONE',  ( 0.000000000000000000, 0.000000000000000000, 1.000000000000000000 ) ) ;
#95941=FACE_OUTER_BOUND ( 'NONE', #10934, .T. ) ;
#95942=CARTESIAN_POINT ( 'NONE',  ( 12.49999999999990585, 12.50000000000000000, -5.022947341949754119 ) ) ;
#95943=CARTESIAN_POINT ( 'NONE',  ( -0.8500000000000395017, 12.50000000000000000, 2.230156782645134950 ) ) ;
#95944=DIRECTION ( 'NONE',  ( 0.000000000000000000, -0.000000000000000000, 1.000000000000000000 ) ) ;
#95945=CARTESIAN_POINT ( 'NONE',  ( -6.250000000000015987, 2.500000000000000000, 1.472243186433545459 ) ) ;
#95946=DIRECTION ( 'NONE',  ( -0.000000000000000000, 1.000000000000000000, -0.000000000000000000 ) ) ;
#95947=VECTOR ( 'NONE', #845, 1000.000000000000000 ) ;
#95948=FACE_OUTER_BOUND ( 'NONE', #119958, .T. ) ;
#95949=EDGE_LOOP ( 'NONE', ( #65199, #112918 ) ) ;
#95951=ORIENTED_EDGE ( 'NONE', *, *, #48756, .T. ) ;
#95952=ORIENTED_EDGE ( 'NONE', *, *, #8188, .F. ) ;
#95953=ORIENTED_EDGE ( 'NONE', *, *, #78265, .F. ) ;
#95954=CONICAL_SURFACE ( 'NONE', #72881, 0.1000000000000000472, 0.003490658503988666988 ) ;
#95955=CARTESIAN_POINT ( 'NONE',  ( -11.64999999999999680, 12.50000000000000000, -2.165063509461097713 ) ) ;
#95956=DIRECTION ( 'NONE',  ( -0.000000000000000000, -1.000000000000000000, -0.000000000000000000 ) ) ;
#95957=EDGE_LOOP ( 'NONE', ( #85243, #15101 ) ) ;
#95958=FACE_BOUND ( 'NONE', #115533, .T. ) ;
#95959=CARTESIAN_POINT ( 'NONE',  ( 0.3999999999999563904, 2.500000000000000000, 5.022947341949748790 ) ) ;
#95960=EDGE_CURVE ( 'NONE', #86833, #106745, #91138, .T. ) ;
#95961=AXIS2_PLACEMENT_3D ( 'NONE', #70441, #17449, #10233 ) ;
#95963=LINE ( 'NONE', #16730, #126821 ) ;
#95964=DIRECTION ( 'NONE',  ( 0.000000000000000000, 0.000000000000000000, -1.000000000000000000 ) ) ;
#95965=EDGE_CURVE ( 'NONE', #91963, #101677, #120195, .T. ) ;
#95966=DIRECTION ( 'NONE',  ( -0.000000000000000000, -1.000000000000000000, -0.000000000000000000 ) ) ;
#95967=ORIENTED_EDGE ( 'NONE', *, *, #17145, .F. ) ;
#95968=VECTOR ( 'NONE', #117394, 1000.000000000000000 ) ;
#95970=EDGE_CURVE ( 'NONE', #110892, #120440, #41411, .T. ) ;
#95971=CONICAL_SURFACE ( 'NONE', #39574, 0.1000000000000002554, 0.003490658503988666988 ) ;
#95972=ORIENTED_EDGE ( 'NONE', *, *, #96119, .F. ) ;
#95973=ORIENTED_EDGE ( 'NONE', *, *, #17769, .T. ) ;
#95974=EDGE_LOOP ( 'NONE', ( #128915, #6232 ) ) ;
#95975=EDGE_CURVE ( 'NONE', #24259, #69008, #17770, .T. ) ;
#95976=LINE ( 'NONE', #62351, #109087 ) ;
#95977=CARTESIAN_POINT ( 'NONE',  ( 3.149999999999944400, 2.500000000000000000, 2.611473670974873151 ) ) ;
#95978=ADVANCED_FACE ( 'NONE', ( #99681 ), #100319, .T. ) ;
#95979=FACE_OUTER_BOUND ( 'NONE', #54055, .T. ) ;
#95980=AXIS2_PLACEMENT_3D ( 'NONE', #101798, #80869, #122083 ) ;
#95981=ADVANCED_FACE ( 'NONE', ( #21100 ), #111875, .T. ) ;
#95982=EDGE_LOOP ( 'NONE', ( #85118, #92758 ) ) ;
#95983=CARTESIAN_POINT ( 'NONE',  ( 13.80955901367088146, 1.499999999999681366, -7.955427458311461031 ) ) ;
#95984=ADVANCED_FACE ( 'NONE', ( #80028 ), #819, .T. ) ;
#95985=CARTESIAN_POINT ( 'NONE',  ( 3.299999999999944755, 2.500000000000000000, -0.1000000000000023925 ) ) ;
#95986=CIRCLE ( 'NONE', #87561, 0.06509327318403745899 ) ;
#95987=CARTESIAN_POINT ( 'NONE',  ( -6.450000000000016165, 12.50000000000000000, 6.841600689897072485 ) ) ;
#95988=VECTOR ( 'NONE', #4459, 1000.000000000000000 ) ;
#95989=EDGE_CURVE ( 'NONE', #11815, #109349, #128622, .T. ) ;
#95991=CARTESIAN_POINT ( 'NONE',  ( -5.650000000000019895, 12.50000000000000000, 6.148780366869520009 ) ) ;
#95992=AXIS2_PLACEMENT_3D ( 'NONE', #60572, #41577, #101768 ) ;
#95993=DIRECTION ( 'NONE',  ( 0.000000000000000000, 0.000000000000000000, 1.000000000000000000 ) ) ;
#95994=EDGE_LOOP ( 'NONE', ( #125140, #49722, #120362, #35748 ) ) ;
#95995=DIRECTION ( 'NONE',  ( -0.000000000000000000, -1.000000000000000000, -0.000000000000000000 ) ) ;
#95996=EDGE_CURVE ( 'NONE', #102123, #56648, #122348, .T. ) ;
#95997=CONICAL_SURFACE ( 'NONE', #16547, 0.1000000000000000472, 0.003490658503988666988 ) ;
#95998=CONICAL_SURFACE ( 'NONE', #100206, 0.1000000000000000472, 0.003490658503988666988 ) ;
#95999=ORIENTED_EDGE ( 'NONE', *, *, #5613, .T. ) ;
#96000=ORIENTED_EDGE ( 'NONE', *, *, #65350, .F. ) ;
#96002=DIRECTION ( 'NONE',  ( 0.000000000000000000, 1.000000000000000000, 0.000000000000000000 ) ) ;
#96003=DIRECTION ( 'NONE',  ( 0.000000000000000000, 0.000000000000000000, -1.000000000000000000 ) ) ;
#96004=ORIENTED_EDGE ( 'NONE', *, *, #16163, .T. ) ;
#96005=ORIENTED_EDGE ( 'NONE', *, *, #109585, .T. ) ;
#96006=CARTESIAN_POINT ( 'NONE',  ( -10.84999999999999964, 2.500000000000000000, 1.472243186433545459 ) ) ;
#96007=LINE ( 'NONE', #7613, #122637 ) ;
#96008=LINE ( 'NONE', #114985, #69057 ) ;
#96009=VECTOR ( 'NONE', #115412, 1000.000000000000000 ) ;
#96010=ORIENTED_EDGE ( 'NONE', *, *, #102587, .F. ) ;
#96011=ORIENTED_EDGE ( 'NONE', *, *, #105846, .F. ) ;
#96012=LINE ( 'NONE', #84898, #33150 ) ;
#96013=ORIENTED_EDGE ( 'NONE', *, *, #50915, .F. ) ;
#96014=CARTESIAN_POINT ( 'NONE',  ( 11.04999999999991189, 2.500000000000000000, 6.148780366869520897 ) ) ;
#96015=CONICAL_SURFACE ( 'NONE', #81364, 0.09999999999999982514, 0.003490658503988666988 ) ;
#96016=CARTESIAN_POINT ( 'NONE',  ( -13.34999999999999076, 12.50000000000000000, -1.537336459617585360 ) ) ;
#96017=VERTEX_POINT ( 'NONE', #129158 ) ;
#96018=CARTESIAN_POINT ( 'NONE',  ( -10.20000000000000462, 12.50000000000000000, 0.2813168883297361700 ) ) ;
#96019=CARTESIAN_POINT ( 'NONE',  ( 13.09999999999990195, 2.500000000000000000, 4.676537180435972552 ) ) ;
#96020=DIRECTION ( 'NONE',  ( 0.000000000000000000, -0.9999939076577903929, 0.003490651415223739937 ) ) ;
#96021=FACE_OUTER_BOUND ( 'NONE', #32751, .T. ) ;
#96022=ORIENTED_EDGE ( 'NONE', *, *, #32603, .F. ) ;
#96023=CONICAL_SURFACE ( 'NONE', #20810, 0.1000000000000000472, 0.003490658503988666988 ) ;
#96024=FACE_OUTER_BOUND ( 'NONE', #14166, .T. ) ;
#96025=EDGE_CURVE ( 'NONE', #97422, #108453, #44982, .T. ) ;
#96026=CARTESIAN_POINT ( 'NONE',  ( 1.049999999999954525, 2.500000000000000000, -2.511473670974877948 ) ) ;
#96027=ORIENTED_EDGE ( 'NONE', *, *, #91953, .T. ) ;
#96028=ORIENTED_EDGE ( 'NONE', *, *, #122922, .F. ) ;
#96029=DIRECTION ( 'NONE',  ( 0.000000000000000000, 0.000000000000000000, 1.000000000000000000 ) ) ;
#96030=CARTESIAN_POINT ( 'NONE',  ( -14.79999999999998295, 12.50000000000000000, -0.2813168883297386680 ) ) ;
#96031=DIRECTION ( 'NONE',  ( 0.000000000000000000, 1.000000000000000000, 0.000000000000000000 ) ) ;
#96032=CARTESIAN_POINT ( 'NONE',  ( 5.849999999999933031, 2.500000000000000000, 7.188010851410848723 ) ) ;
#96033=DIRECTION ( 'NONE',  ( 0.000000000000000000, 0.000000000000000000, -1.000000000000000000 ) ) ;
#96034=DIRECTION ( 'NONE',  ( 0.000000000000000000, 1.000000000000000000, 0.000000000000000000 ) ) ;
#96035=EDGE_CURVE ( 'NONE', #89842, #44383, #113930, .T. ) ;
#96036=AXIS2_PLACEMENT_3D ( 'NONE', #79488, #90575, #100408 ) ;
#96037=AXIS2_PLACEMENT_3D ( 'NONE', #98323, #129116, #8644 ) ;
#96038=CARTESIAN_POINT ( 'NONE',  ( -2.700000000000030820, 12.50000000000000000, 0.4115034346978109769 ) ) ;
#96039=FACE_OUTER_BOUND ( 'NONE', #96101, .T. ) ;
#96040=CARTESIAN_POINT ( 'NONE',  ( -1.650000000000035216, 2.500000000000000000, -5.802370205355749988 ) ) ;
#96041=CARTESIAN_POINT ( 'NONE',  ( 13.34999999999989662, 2.500000000000000000, -2.165063509461101710 ) ) ;
#96042=ORIENTED_EDGE ( 'NONE', *, *, #24860, .F. ) ;
#96043=ORIENTED_EDGE ( 'NONE', *, *, #84283, .F. ) ;
#96044=CARTESIAN_POINT ( 'NONE',  ( -15.39999999999997904, 2.500000000000000000, -0.5928203230275518321 ) ) ;
#96045=EDGE_LOOP ( 'NONE', ( #35770, #120380, #61798, #43468 ) ) ;
#96046=CARTESIAN_POINT ( 'NONE',  ( 10.39999999999991154, 12.50000000000000000, 5.088040615133786027 ) ) ;
#96047=DIRECTION ( 'NONE',  ( 0.000000000000000000, 0.000000000000000000, 1.000000000000000000 ) ) ;
#96048=DIRECTION ( 'NONE',  ( -0.000000000000000000, -1.000000000000000000, -0.000000000000000000 ) ) ;
#96049=VERTEX_POINT ( 'NONE', #59773 ) ;
#96050=CARTESIAN_POINT ( 'NONE',  ( 17.79089025268834590, -2.511997385349132195, -2.795007471442499725 ) ) ;
#96051=CARTESIAN_POINT ( 'NONE',  ( 6.049999999999932321, 2.500000000000000000, 1.918653347947321564 ) ) ;
#96052=CARTESIAN_POINT ( 'NONE',  ( 12.04999999999990834, 2.500000000000000000, -2.065063509461102065 ) ) ;
#96053=VERTEX_POINT ( 'NONE', #74073 ) ;
#96055=VECTOR ( 'NONE', #66871, 1000.000000000000000 ) ;
#96056=CARTESIAN_POINT ( 'NONE',  ( -1.450000000000036371, 12.50000000000000000, 6.906693963081109722 ) ) ;
#96057=EDGE_LOOP ( 'NONE', ( #74567, #127396 ) ) ;
#96058=EDGE_CURVE ( 'NONE', #61588, #45891, #84535, .T. ) ;
#96059=EDGE_LOOP ( 'NONE', ( #123876, #60392, #13644, #110006 ) ) ;
#96060=VERTEX_POINT ( 'NONE', #42044 ) ;
#96061=EDGE_LOOP ( 'NONE', ( #52851, #60053, #14135, #11925 ) ) ;
#96062=CARTESIAN_POINT ( 'NONE',  ( -11.24999999999996447, 2.500000000000000000, -6.595190528383298556 ) ) ;
#96063=CIRCLE ( 'NONE', #110645, 0.06509327318403745899 ) ;
#96064=DIRECTION ( 'NONE',  ( -0.000000000000000000, 1.000000000000000000, -0.000000000000000000 ) ) ;
#96066=CARTESIAN_POINT ( 'NONE',  ( -9.350000000000004974, 12.50000000000000000, 6.841600689897072485 ) ) ;
#96067=ADVANCED_FACE ( 'NONE', ( #62333 ), #123184, .T. ) ;
#96068=EDGE_LOOP ( 'NONE', ( #36567, #100322 ) ) ;
#96069=CIRCLE ( 'NONE', #27033, 0.1000000000000002554 ) ;
#96070=VECTOR ( 'NONE', #449, 1000.000000000000000 ) ;
#96071=CARTESIAN_POINT ( 'NONE',  ( -6.650000000000018119, 12.50000000000000000, -6.495190528383302464 ) ) ;
#96072=VERTEX_POINT ( 'NONE', #33520 ) ;
#96073=DIRECTION ( 'NONE',  ( 0.000000000000000000, 0.000000000000000000, -1.000000000000000000 ) ) ;
#96074=DIRECTION ( 'NONE',  ( 0.000000000000000000, 0.000000000000000000, -1.000000000000000000 ) ) ;
#96075=VECTOR ( 'NONE', #78110, 1000.000000000000000 ) ;
#96076=EDGE_CURVE ( 'NONE', #124065, #68389, #118118, .T. ) ;
#96077=CARTESIAN_POINT ( 'NONE',  ( -10.20000000000000462, 2.500000000000000000, 4.576537180435972019 ) ) ;
#96078=CARTESIAN_POINT ( 'NONE',  ( 18.37149739119674052, -2.540880845002044808, 2.596776292461127067 ) ) ;
#96079=EDGE_CURVE ( 'NONE', #9068, #29188, #65887, .T. ) ;
#96082=VECTOR ( 'NONE', #97207, 1000.000000000000000 ) ;
#96083=ORIENTED_EDGE ( 'NONE', *, *, #117350, .F. ) ;
#96084=EDGE_CURVE ( 'NONE', #111361, #105503, #88879, .T. ) ;
#96085=ORIENTED_EDGE ( 'NONE', *, *, #107250, .T. ) ;
#96086=DIRECTION ( 'NONE',  ( 0.000000000000000000, 0.000000000000000000, 1.000000000000000000 ) ) ;
#96087=CARTESIAN_POINT ( 'NONE',  ( -8.750000000000010658, 2.500000000000000000, -1.572243186433550211 ) ) ;
#96088=CARTESIAN_POINT ( 'NONE',  ( 7.099999999999925926, 12.50000000000000000, 0.7579135962115869374 ) ) ;
#96089=ADVANCED_FACE ( 'NONE', ( #22419 ), #3118, .T. ) ;
#96090=FACE_BOUND ( 'NONE', #87454, .T. ) ;
#96091=CARTESIAN_POINT ( 'NONE',  ( 5.199999999999933564, 2.500000000000000000, 3.983716857408420076 ) ) ;
#96092=DIRECTION ( 'NONE',  ( -0.000000000000000000, 1.000000000000000000, -0.000000000000000000 ) ) ;
#96093=CARTESIAN_POINT ( 'NONE',  ( -3.470671598752761919E-14, 2.500000000000000000, -0.7928203230275518987 ) ) ;
#96094=FACE_OUTER_BOUND ( 'NONE', #76415, .T. ) ;
#96096=CARTESIAN_POINT ( 'NONE',  ( -11.44999999999999751, 2.500000000000000000, 1.818653347947321475 ) ) ;
#96097=CARTESIAN_POINT ( 'NONE',  ( -12.89999999999999147, 12.50000000000000000, 4.395220292106234439 ) ) ;
#96098=VECTOR ( 'NONE', #111275, 1000.000000000000000 ) ;
#96099=AXIS2_PLACEMENT_3D ( 'NONE', #5712, #115670, #115022 ) ;
#96100=FACE_OUTER_BOUND ( 'NONE', #8485, .T. ) ;
#96101=EDGE_LOOP ( 'NONE', ( #70438, #118126 ) ) ;
#96102=ORIENTED_EDGE ( 'NONE', *, *, #89631, .T. ) ;
#96103=ORIENTED_EDGE ( 'NONE', *, *, #92242, .F. ) ;
#96104=VERTEX_POINT ( 'NONE', #104175 ) ;
#96105=LINE ( 'NONE', #94822, #21473 ) ;
#96106=FACE_BOUND ( 'NONE', #74147, .T. ) ;
#96107=DIRECTION ( 'NONE',  ( 0.000000000000000000, 0.000000000000000000, 1.000000000000000000 ) ) ;
#96108=VECTOR ( 'NONE', #87322, 1000.000000000000000 ) ;
#96109=VECTOR ( 'NONE', #87777, 1000.000000000000000 ) ;
#96110=DIRECTION ( 'NONE',  ( 0.000000000000000000, 0.000000000000000000, 1.000000000000000000 ) ) ;
#96111=EDGE_LOOP ( 'NONE', ( #45771, #122710 ) ) ;
#96112=CARTESIAN_POINT ( 'NONE',  ( -12.29999999999999538, 2.500000000000000000, -0.4464101615137742174 ) ) ;
#96113=CARTESIAN_POINT ( 'NONE',  ( 14.14999999999989733, 12.50000000000000000, 2.922977105672686982 ) ) ;
#96114=ORIENTED_EDGE ( 'NONE', *, *, #65929, .F. ) ;
#96115=DIRECTION ( 'NONE',  ( 0.000000000000000000, 0.000000000000000000, 1.000000000000000000 ) ) ;
#96116=FACE_OUTER_BOUND ( 'NONE', #117357, .T. ) ;
#96117=AXIS2_PLACEMENT_3D ( 'NONE', #37480, #64973, #65625 ) ;
#96118=CONICAL_SURFACE ( 'NONE', #104534, 0.09999999999999999167, 0.003490658503988666988 ) ;
#96119=EDGE_CURVE ( 'NONE', #9837, #66463, #59579, .T. ) ;
#96120=ORIENTED_EDGE ( 'NONE', *, *, #79669, .F. ) ;
#96121=EDGE_CURVE ( 'NONE', #104198, #25500, #128720, .T. ) ;
#96122=FACE_OUTER_BOUND ( 'NONE', #122958, .T. ) ;
#96123=DIRECTION ( 'NONE',  ( 0.000000000000000000, -0.000000000000000000, 1.000000000000000000 ) ) ;
#96124=EDGE_CURVE ( 'NONE', #79633, #66106, #101504, .T. ) ;
#96125=VECTOR ( 'NONE', #106063, 1000.000000000000000 ) ;
#96126=EDGE_CURVE ( 'NONE', #32665, #120157, #76461, .T. ) ;
#96127=VERTEX_POINT ( 'NONE', #81950 ) ;
#96128=LINE ( 'NONE', #116404, #82324 ) ;
#96129=CARTESIAN_POINT ( 'NONE',  ( -5.800000000000022027, 2.500000000000000000, -4.330127018922201643 ) ) ;
#96130=EDGE_LOOP ( 'NONE', ( #122956, #55945 ) ) ;
#96131=LINE ( 'NONE', #96764, #72356 ) ;
#96132=ADVANCED_FACE ( 'NONE', ( #21761 ), #38832, .T. ) ;
#96133=ORIENTED_EDGE ( 'NONE', *, *, #93035, .T. ) ;
#96135=CARTESIAN_POINT ( 'NONE',  ( -2.950000000000033484, 12.50000000000000000, -6.495190528383302464 ) ) ;
#96136=VERTEX_POINT ( 'NONE', #44615 ) ;
#96137=DIRECTION ( 'NONE',  ( 0.000000000000000000, 1.000000000000000000, 0.000000000000000000 ) ) ;
#96138=FACE_BOUND ( 'NONE', #91117, .T. ) ;
#96139=EDGE_CURVE ( 'NONE', #26496, #60288, #126543, .T. ) ;
#96140=EDGE_CURVE ( 'NONE', #1757, #72027, #34818, .T. ) ;
#96141=EDGE_LOOP ( 'NONE', ( #70186, #65641 ) ) ;
#96142=CARTESIAN_POINT ( 'NONE',  ( -10.40000000000000213, 2.500000000000000000, -0.6928203230275541413 ) ) ;
#96143=CARTESIAN_POINT ( 'NONE',  ( -9.600000000000008527, 12.50000000000000000, -4.265033745738159965 ) ) ;
#96144=DIRECTION ( 'NONE',  ( 0.000000000000000000, 0.000000000000000000, 1.000000000000000000 ) ) ;
#96145=FACE_OUTER_BOUND ( 'NONE', #125563, .T. ) ;
#96146=CARTESIAN_POINT ( 'NONE',  ( -2.100000000000033396, 12.50000000000000000, -0.6928203230275542523 ) ) ;
#96147=DIRECTION ( 'NONE',  ( 0.000000000000000000, 0.000000000000000000, 1.000000000000000000 ) ) ;
#96148=ORIENTED_EDGE ( 'NONE', *, *, #64793, .T. ) ;
#96149=ORIENTED_EDGE ( 'NONE', *, *, #91412, .T. ) ;
#96150=CARTESIAN_POINT ( 'NONE',  ( -1.850000000000033396, 2.500000000000000000, -2.511473670974877948 ) ) ;
#96151=CARTESIAN_POINT ( 'NONE',  ( -6.050000000000017586, 2.500000000000000000, 1.818653347947321475 ) ) ;
#96152=CARTESIAN_POINT ( 'NONE',  ( -1.650000000000034772, 2.500000000000000000, 2.265063509461097357 ) ) ;
#96153=ORIENTED_EDGE ( 'NONE', *, *, #122852, .F. ) ;
#96154=EDGE_LOOP ( 'NONE', ( #120841, #106250, #60405, #43309 ) ) ;
#96155=ORIENTED_EDGE ( 'NONE', *, *, #119006, .T. ) ;
#96156=CONICAL_SURFACE ( 'NONE', #108675, 0.1000000000000000472, 0.003490658503988666988 ) ;
#96157=CARTESIAN_POINT ( 'NONE',  ( -14.34999999999998543, 2.500000000000000000, -2.411473670974875638 ) ) ;
#96158=CARTESIAN_POINT ( 'NONE',  ( -4.350000000000023626, 2.500000000000000000, 6.148780366869520897 ) ) ;
#96159=DIRECTION ( 'NONE',  ( 0.000000000000000000, -0.9999939076577903929, 0.003490651415223739937 ) ) ;
#96160=AXIS2_PLACEMENT_3D ( 'NONE', #118756, #6206, #58565 ) ;
#96161=PLANE ( 'NONE',  #64094 ) ;
#96162=CARTESIAN_POINT ( 'NONE',  ( -6.850000000000017408, 2.500000000000000000, -6.941600689897077459 ) ) ;
#96163=CARTESIAN_POINT ( 'NONE',  ( -14.79999999999998472, 2.500000000000000000, 0.2464101615137758439 ) ) ;
#96164=CARTESIAN_POINT ( 'NONE',  ( -10.80000000000000071, 2.500000000000000000, -2.276824562219559311E-15 ) ) ;
#96165=DIRECTION ( 'NONE',  ( 0.000000000000000000, 0.000000000000000000, 1.000000000000000000 ) ) ;
#96166=LINE ( 'NONE', #29385, #18568 ) ;
#96167=AXIS2_PLACEMENT_3D ( 'NONE', #39300, #87705, #18959 ) ;
#96168=ORIENTED_EDGE ( 'NONE', *, *, #121294, .T. ) ;
#96169=CARTESIAN_POINT ( 'NONE',  ( 8.149999999999920419, 12.50000000000000000, -2.576566944158915184 ) ) ;
#96170=VERTEX_POINT ( 'NONE', #23044 ) ;
#96171=ORIENTED_EDGE ( 'NONE', *, *, #98641, .T. ) ;
#96172=CARTESIAN_POINT ( 'NONE',  ( -6.250000000000019540, 12.50000000000000000, -2.857883832488653741 ) ) ;
#96173=CARTESIAN_POINT ( 'NONE',  ( 9.149999999999918643, 2.500000000000000000, 2.165063509461097713 ) ) ;
#96174=CARTESIAN_POINT ( 'NONE',  ( -6.650000000000014566, 2.500000000000000000, 5.902370205355745192 ) ) ;
#96175=LINE ( 'NONE', #45809, #117381 ) ;
#96176=EDGE_CURVE ( 'NONE', #87768, #54395, #9560, .T. ) ;
#96177=DIRECTION ( 'NONE',  ( 0.000000000000000000, 1.000000000000000000, 0.000000000000000000 ) ) ;
#96178=DIRECTION ( 'NONE',  ( -0.000000000000000000, -1.000000000000000000, -0.000000000000000000 ) ) ;
#96179=CARTESIAN_POINT ( 'NONE',  ( -12.89999999999999325, 2.500000000000000000, 0.5928203230275536084 ) ) ;
#96180=VERTEX_POINT ( 'NONE', #83881 ) ;
#96182=DIRECTION ( 'NONE',  ( 0.000000000000000000, -0.9999939076577903929, 0.003490651415223739937 ) ) ;
#96183=ORIENTED_EDGE ( 'NONE', *, *, #85309, .F. ) ;
#96185=AXIS2_PLACEMENT_3D ( 'NONE', #106912, #68930, #18542 ) ;
#96186=ORIENTED_EDGE ( 'NONE', *, *, #77795, .F. ) ;
#96187=EDGE_LOOP ( 'NONE', ( #105871, #897, #71665, #17878 ) ) ;
#96188=ORIENTED_EDGE ( 'NONE', *, *, #55455, .F. ) ;
#96189=DIRECTION ( 'NONE',  ( 0.000000000000000000, 0.000000000000000000, -1.000000000000000000 ) ) ;
#96190=CARTESIAN_POINT ( 'NONE',  ( -4.294665249841745289E-14, 2.500000000000000000, 4.922947341949748257 ) ) ;
#96191=CIRCLE ( 'NONE', #39795, 0.06509327318403745899 ) ;
#96192=VERTEX_POINT ( 'NONE', #2745 ) ;
#96193=CARTESIAN_POINT ( 'NONE',  ( 14.34999999999989662, 2.500000000000000000, 1.818653347947321475 ) ) ;
#96194=CARTESIAN_POINT ( 'NONE',  ( 17.50000000000000000, -0.9166666666666695162, -3.432456362931489036 ) ) ;
#96195=CARTESIAN_POINT ( 'NONE',  ( 5.399999999999935518, 2.500000000000000000, -4.330127018922201643 ) ) ;
#96196=ORIENTED_EDGE ( 'NONE', *, *, #70517, .T. ) ;
#96197=DIRECTION ( 'NONE',  ( 0.000000000000000000, 0.000000000000000000, 1.000000000000000000 ) ) ;
#96198=AXIS2_PLACEMENT_3D ( 'NONE', #118970, #36065, #128828 ) ;
#96199=CARTESIAN_POINT ( 'NONE',  ( 12.89999999999989910, 2.500000000000000000, 0.6928203230275494784 ) ) ;
#96200=CIRCLE ( 'NONE', #41948, 0.06509327318403745899 ) ;
#96201=ORIENTED_EDGE ( 'NONE', *, *, #17149, .T. ) ;
#96202=CONICAL_SURFACE ( 'NONE', #10526, 0.1000000000000002554, 0.003490658503988666988 ) ;
#96203=EDGE_LOOP ( 'NONE', ( #45879, #98788, #117034, #98381 ) ) ;
#96204=VERTEX_POINT ( 'NONE', #42711 ) ;
#96205=FACE_OUTER_BOUND ( 'NONE', #119294, .T. ) ;
#96206=AXIS2_PLACEMENT_3D ( 'NONE', #90268, #128952, #50364 ) ;
#96207=PLANE ( 'NONE',  #108811 ) ;
#96208=ADVANCED_FACE ( 'NONE', ( #13852 ), #82620, .T. ) ;
#96209=CONICAL_SURFACE ( 'NONE', #108743, 0.1000000000000002554, 0.003490658503988666988 ) ;
#96210=ORIENTED_EDGE ( 'NONE', *, *, #67722, .F. ) ;
#96211=DIRECTION ( 'NONE',  ( 0.000000000000000000, 0.000000000000000000, 1.000000000000000000 ) ) ;
#96212=DIRECTION ( 'NONE',  ( 0.000000000000000000, -0.000000000000000000, 1.000000000000000000 ) ) ;
#96213=EDGE_CURVE ( 'NONE', #105627, #1738, #88977, .T. ) ;
#96214=CARTESIAN_POINT ( 'NONE',  ( -7.100000000000014744, 2.500000000000000000, 4.330127018922196314 ) ) ;
#96215=FACE_OUTER_BOUND ( 'NONE', #125248, .T. ) ;
#96216=EDGE_CURVE ( 'NONE', #119760, #8618, #13652, .T. ) ;
#96217=ORIENTED_EDGE ( 'NONE', *, *, #121865, .F. ) ;
#96218=DIRECTION ( 'NONE',  ( 0.000000000000000000, 0.000000000000000000, 1.000000000000000000 ) ) ;
#96219=ORIENTED_EDGE ( 'NONE', *, *, #71905, .F. ) ;
#96220=ADVANCED_FACE ( 'NONE', ( #114629 ), #55715, .T. ) ;
#96221=ADVANCED_FACE ( 'NONE', ( #7242 ), #19934, .T. ) ;
#96222=EDGE_LOOP ( 'NONE', ( #118522, #63154 ) ) ;
#96223=VERTEX_POINT ( 'NONE', #87742 ) ;
#96224=EDGE_CURVE ( 'NONE', #89145, #3186, #17041, .T. ) ;
#96225=CARTESIAN_POINT ( 'NONE',  ( 10.64999999999990976, 2.500000000000000000, 2.411473670974873862 ) ) ;
#96226=EDGE_CURVE ( 'NONE', #44658, #21383, #70112, .T. ) ;
#96227=ADVANCED_FACE ( 'NONE', ( #46530 ), #51345, .T. ) ;
#96228=FACE_BOUND ( 'NONE', #8075, .T. ) ;
#96229=CARTESIAN_POINT ( 'NONE',  ( -7.500000000000011546, 12.50000000000000000, 3.572213422710607489 ) ) ;
#96230=CARTESIAN_POINT ( 'NONE',  ( 2.899999999999945732, 12.50000000000000000, -2.385244779468109755E-15 ) ) ;
#96231=CARTESIAN_POINT ( 'NONE',  ( 7.499999999999925393, 12.50000000000000000, 4.957854068765711553 ) ) ;
#96232=AXIS2_PLACEMENT_3D ( 'NONE', #42255, #42921, #31158 ) ;
#96233=ORIENTED_EDGE ( 'NONE', *, *, #99926, .T. ) ;
#96235=CONICAL_SURFACE ( 'NONE', #115020, 0.1000000000000000472, 0.003490658503988666988 ) ;
#96237=EDGE_CURVE ( 'NONE', #117173, #19230, #93101, .T. ) ;
#96238=DIRECTION ( 'NONE',  ( 0.000000000000000000, 1.000000000000000000, 0.000000000000000000 ) ) ;
#96239=LINE ( 'NONE', #77262, #57319 ) ;
#96240=ORIENTED_EDGE ( 'NONE', *, *, #104277, .T. ) ;
#96241=CARTESIAN_POINT ( 'NONE',  ( -3.350000000000028511, 12.50000000000000000, -1.472243186433550122 ) ) ;
#96242=CONICAL_SURFACE ( 'NONE', #27201, 0.1000000000000002554, 0.003490658503988666988 ) ;
#96243=DIRECTION ( 'NONE',  ( 0.000000000000000000, 0.000000000000000000, 1.000000000000000000 ) ) ;
#96244=EDGE_LOOP ( 'NONE', ( #112866, #61347, #19194, #87832 ) ) ;
#96245=CARTESIAN_POINT ( 'NONE',  ( 2.099999999999947686, 2.500000000000000000, 5.022947341949748790 ) ) ;
#96246=CARTESIAN_POINT ( 'NONE',  ( -1.850000000000033396, 12.50000000000000000, -6.906693963081115051 ) ) ;
#96247=FACE_BOUND ( 'NONE', #88740, .T. ) ;
#96249=ORIENTED_EDGE ( 'NONE', *, *, #74995, .T. ) ;
#96250=CARTESIAN_POINT ( 'NONE',  ( 4.149999999999936406, 12.50000000000000000, 6.430097255199259010 ) ) ;
#96251=CARTESIAN_POINT ( 'NONE',  ( -3.950000000000025491, 2.500000000000000000, 6.248780366869521430 ) ) ;
#96252=VERTEX_POINT ( 'NONE', #36743 ) ;
#96253=ORIENTED_EDGE ( 'NONE', *, *, #120084, .F. ) ;
#96255=ORIENTED_EDGE ( 'NONE', *, *, #78669, .F. ) ;
#96257=DIRECTION ( 'NONE',  ( 0.000000000000000000, 0.000000000000000000, -1.000000000000000000 ) ) ;
#96258=CARTESIAN_POINT ( 'NONE',  ( 5.599999999999931255, 12.50000000000000000, 4.676537180435972552 ) ) ;
#96259=DIRECTION ( 'NONE',  ( 0.000000000000000000, 0.000000000000000000, -1.000000000000000000 ) ) ;
#96260=EDGE_CURVE ( 'NONE', #92915, #86749, #3216, .T. ) ;
#96261=EDGE_CURVE ( 'NONE', #49329, #2409, #68038, .T. ) ;
#96262=CARTESIAN_POINT ( 'NONE',  ( -9.550000000000006040, 12.50000000000000000, -2.165063509461101710 ) ) ;
#96263=ADVANCED_FACE ( 'NONE', ( #115926 ), #37383, .T. ) ;
#96264=CONICAL_SURFACE ( 'NONE', #75343, 0.1000000000000002554, 0.003490658503988666988 ) ;
#96265=AXIS2_PLACEMENT_3D ( 'NONE', #9076, #30677, #11654 ) ;
#96266=EDGE_LOOP ( 'NONE', ( #26532, #105914, #91804, #38753 ) ) ;
#96267=EDGE_CURVE ( 'NONE', #120717, #114882, #26906, .T. ) ;
#96268=DIRECTION ( 'NONE',  ( 0.000000000000000000, 0.000000000000000000, 1.000000000000000000 ) ) ;
#96269=CARTESIAN_POINT ( 'NONE',  ( 2.500000000000002220, -2.500000000000000000, -8.999999999999998224 ) ) ;
#96270=LINE ( 'NONE', #6579, #61799 ) ;
#96271=LINE ( 'NONE', #96924, #13505 ) ;
#96272=ORIENTED_EDGE ( 'NONE', *, *, #43511, .T. ) ;
#96273=VERTEX_POINT ( 'NONE', #117182 ) ;
#96274=FACE_BOUND ( 'NONE', #124881, .T. ) ;
#96275=ORIENTED_EDGE ( 'NONE', *, *, #28438, .F. ) ;
#96276=EDGE_CURVE ( 'NONE', #585, #48425, #11605, .T. ) ;
#96277=DIRECTION ( 'NONE',  ( 0.000000000000000000, 0.000000000000000000, 1.000000000000000000 ) ) ;
#96278=DIRECTION ( 'NONE',  ( 0.000000000000000000, 1.000000000000000000, 0.000000000000000000 ) ) ;
#96279=VECTOR ( 'NONE', #47625, 1000.000000000000000 ) ;
#96280=EDGE_CURVE ( 'NONE', #30789, #81006, #26290, .T. ) ;
#96281=VERTEX_POINT ( 'NONE', #24970 ) ;
#96282=LINE ( 'NONE', #67451, #5129 ) ;
#96283=CARTESIAN_POINT ( 'NONE',  ( 87.50000000000001421, -3.974992050023848922, -6.359987280038160051 ) ) ;
#96284=EDGE_CURVE ( 'NONE', #113131, #110912, #24140, .T. ) ;
#96285=CARTESIAN_POINT ( 'NONE',  ( -6.450000000000016165, 2.500000000000000000, 6.841600689897072485 ) ) ;
#96286=ADVANCED_FACE ( 'NONE', ( #96923 ), #45911, .T. ) ;
#96287=CARTESIAN_POINT ( 'NONE',  ( -10.84999999999999964, 12.50000000000000000, 2.857883832488649301 ) ) ;
#96288=ORIENTED_EDGE ( 'NONE', *, *, #30866, .T. ) ;
#96289=DIRECTION ( 'NONE',  ( 0.000000000000000000, -0.9999939076577903929, 0.003490651415223739937 ) ) ;
#96290=CARTESIAN_POINT ( 'NONE',  ( 13.54999999999989591, 2.500000000000000000, -1.918653347947326004 ) ) ;
#96291=CARTESIAN_POINT ( 'NONE',  ( -12.29999999999999538, 12.50000000000000000, 4.676537180435972552 ) ) ;
#96292=DIRECTION ( 'NONE',  ( 0.000000000000000000, 0.000000000000000000, 1.000000000000000000 ) ) ;
#96293=DIRECTION ( 'NONE',  ( -4.274815082592931898E-19, -0.9999939076577903929, -0.003490651415223739937 ) ) ;
#96294=EDGE_CURVE ( 'NONE', #29207, #60583, #36084, .T. ) ;
#96296=ORIENTED_EDGE ( 'NONE', *, *, #39128, .F. ) ;
#96297=AXIS2_PLACEMENT_3D ( 'NONE', #58110, #7042, #96718 ) ;
#96298=ORIENTED_EDGE ( 'NONE', *, *, #93601, .T. ) ;
#96299=DIRECTION ( 'NONE',  ( 0.000000000000000000, 0.000000000000000000, 1.000000000000000000 ) ) ;
#96300=ORIENTED_EDGE ( 'NONE', *, *, #90389, .T. ) ;
#96301=CARTESIAN_POINT ( 'NONE',  ( -10.40000000000000213, 2.500000000000000000, 4.230127018922196669 ) ) ;
#96302=ORIENTED_EDGE ( 'NONE', *, *, #35542, .F. ) ;
#96303=ORIENTED_EDGE ( 'NONE', *, *, #68874, .T. ) ;
#96304=ORIENTED_EDGE ( 'NONE', *, *, #52989, .T. ) ;
#96305=CARTESIAN_POINT ( 'NONE',  ( -14.34999999999998543, 12.50000000000000000, -1.883746621131361154 ) ) ;
#96306=AXIS2_PLACEMENT_3D ( 'NONE', #22220, #62136, #42498 ) ;
#96307=DIRECTION ( 'NONE',  ( 0.000000000000000000, 1.000000000000000000, 0.000000000000000000 ) ) ;
#96309=DIRECTION ( 'NONE',  ( -0.000000000000000000, -1.000000000000000000, -0.000000000000000000 ) ) ;
#96310=CIRCLE ( 'NONE', #18939, 0.09999999999999982514 ) ;
#96311=LINE ( 'NONE', #87139, #71075 ) ;
#96312=DIRECTION ( 'NONE',  ( -0.000000000000000000, -1.000000000000000000, -0.000000000000000000 ) ) ;
#96313=EDGE_CURVE ( 'NONE', #108949, #112141, #96270, .T. ) ;
#96314=ORIENTED_EDGE ( 'NONE', *, *, #42513, .F. ) ;
#96315=DIRECTION ( 'NONE',  ( 0.000000000000000000, 1.000000000000000000, 0.000000000000000000 ) ) ;
#96316=ORIENTED_EDGE ( 'NONE', *, *, #54347, .T. ) ;
#96317=ORIENTED_EDGE ( 'NONE', *, *, #45862, .T. ) ;
#96318=ORIENTED_EDGE ( 'NONE', *, *, #10403, .T. ) ;
#96319=ORIENTED_EDGE ( 'NONE', *, *, #29787, .F. ) ;
#96320=DIRECTION ( 'NONE',  ( -4.274815082592931898E-19, -0.9999939076577903929, -0.003490651415223739937 ) ) ;
#96321=ORIENTED_EDGE ( 'NONE', *, *, #47711, .T. ) ;
#96322=VERTEX_POINT ( 'NONE', #87104 ) ;
#96323=DIRECTION ( 'NONE',  ( 0.000000000000000000, 0.000000000000000000, -1.000000000000000000 ) ) ;
#96324=DIRECTION ( 'NONE',  ( -0.000000000000000000, 1.000000000000000000, -0.000000000000000000 ) ) ;
#96325=EDGE_CURVE ( 'NONE', #63506, #104598, #76369, .T. ) ;
#96326=PLANE ( 'NONE',  #92320 ) ;
#96327=CARTESIAN_POINT ( 'NONE',  ( 0.7999999999999553024, 2.500000000000000000, -4.330127018922201643 ) ) ;
#96328=AXIS2_PLACEMENT_3D ( 'NONE', #83476, #53364, #93280 ) ;
#96329=LINE ( 'NONE', #8585, #126153 ) ;
#96330=EDGE_LOOP ( 'NONE', ( #73072, #42798, #86437, #40285 ) ) ;
#96331=AXIS2_PLACEMENT_3D ( 'NONE', #47421, #118076, #69625 ) ;
#96332=AXIS2_PLACEMENT_3D ( 'NONE', #82171, #102457, #92632 ) ;
#96333=LINE ( 'NONE', #60781, #53359 ) ;
#96334=VERTEX_POINT ( 'NONE', #49787 ) ;
#96335=CARTESIAN_POINT ( 'NONE',  ( -0.6500000000000403233, 2.500000000000000000, 6.048780366869520364 ) ) ;
#96337=ORIENTED_EDGE ( 'NONE', *, *, #91890, .T. ) ;
#96338=DIRECTION ( 'NONE',  ( 0.000000000000000000, 0.000000000000000000, -1.000000000000000000 ) ) ;
#96339=EDGE_LOOP ( 'NONE', ( #100609, #81496, #86110, #22883 ) ) ;
#96341=EDGE_CURVE ( 'NONE', #85026, #12477, #77932, .T. ) ;
#96342=ORIENTED_EDGE ( 'NONE', *, *, #101381, .F. ) ;
#96343=DIRECTION ( 'NONE',  ( 0.000000000000000000, 1.000000000000000000, 0.000000000000000000 ) ) ;
#96344=FACE_OUTER_BOUND ( 'NONE', #14903, .T. ) ;
#96345=CARTESIAN_POINT ( 'NONE',  ( -4.293440603042597559E-14, 2.500000000000000000, 5.022947341949748790 ) ) ;
#96346=DIRECTION ( 'NONE',  ( -0.000000000000000000, 1.000000000000000000, -0.000000000000000000 ) ) ;
#96347=DIRECTION ( 'NONE',  ( 0.000000000000000000, 0.000000000000000000, -1.000000000000000000 ) ) ;
#96348=ORIENTED_EDGE ( 'NONE', *, *, #84984, .F. ) ;
#96349=DIRECTION ( 'NONE',  ( 0.000000000000000000, 1.000000000000000000, 0.000000000000000000 ) ) ;
#96350=DIRECTION ( 'NONE',  ( -4.274815082592931898E-19, -0.9999939076577903929, -0.003490651415223739937 ) ) ;
#96351=DIRECTION ( 'NONE',  ( 0.000000000000000000, 0.000000000000000000, -1.000000000000000000 ) ) ;
#96352=DIRECTION ( 'NONE',  ( 0.000000000000000000, 0.000000000000000000, 1.000000000000000000 ) ) ;
#96353=CARTESIAN_POINT ( 'NONE',  ( -0.8500000000000386136, 2.500000000000000000, 2.757883832488649656 ) ) ;
#96354=EDGE_LOOP ( 'NONE', ( #67484, #116185, #122656, #88133 ) ) ;
#96356=ORIENTED_EDGE ( 'NONE', *, *, #90143, .F. ) ;
#96357=CARTESIAN_POINT ( 'NONE',  ( -3.150000000000030109, 2.500000000000000000, 1.718653347947321386 ) ) ;
#96358=ORIENTED_EDGE ( 'NONE', *, *, #47660, .T. ) ;
#96359=DIRECTION ( 'NONE',  ( 0.000000000000000000, 0.000000000000000000, -1.000000000000000000 ) ) ;
#96360=AXIS2_PLACEMENT_3D ( 'NONE', #117110, #77214, #127602 ) ;
#96361=DIRECTION ( 'NONE',  ( -0.000000000000000000, -1.000000000000000000, -0.000000000000000000 ) ) ;
#96362=AXIS2_PLACEMENT_3D ( 'NONE', #48205, #6960, #46263 ) ;
#96363=EDGE_CURVE ( 'NONE', #118657, #27686, #78536, .T. ) ;
#96364=ORIENTED_EDGE ( 'NONE', *, *, #14507, .T. ) ;
#96366=FACE_OUTER_BOUND ( 'NONE', #81061, .T. ) ;
#96367=FACE_OUTER_BOUND ( 'NONE', #31508, .T. ) ;
#96368=CARTESIAN_POINT ( 'NONE',  ( -11.44999999999999751, 2.500000000000000000, -2.611473670974873595 ) ) ;
#96369=CARTESIAN_POINT ( 'NONE',  ( 1.899999999999951283, 12.50000000000000000, -3.983716857408426293 ) ) ;
#96370=ORIENTED_EDGE ( 'NONE', *, *, #98979, .F. ) ;
#96371=EDGE_CURVE ( 'NONE', #52515, #32613, #28343, .T. ) ;
#96372=AXIS2_PLACEMENT_3D ( 'NONE', #129052, #9255, #28904 ) ;
#96373=DIRECTION ( 'NONE',  ( 0.000000000000000000, 1.000000000000000000, 0.000000000000000000 ) ) ;
#96374=CARTESIAN_POINT ( 'NONE',  ( -2.300000000000033129, 12.50000000000000000, 3.983716857408420076 ) ) ;
#96375=ORIENTED_EDGE ( 'NONE', *, *, #14381, .T. ) ;
#96376=EDGE_CURVE ( 'NONE', #40814, #32532, #43034, .T. ) ;
#96377=ADVANCED_FACE ( 'NONE', ( #20953 ), #128352, .T. ) ;
#96378=EDGE_CURVE ( 'NONE', #7910, #110892, #59754, .T. ) ;
#96379=PLANE ( 'NONE',  #48505 ) ;
#96380=EDGE_CURVE ( 'NONE', #125657, #102321, #22095, .T. ) ;
#96381=DIRECTION ( 'NONE',  ( -0.000000000000000000, -1.000000000000000000, -0.000000000000000000 ) ) ;
#96382=CARTESIAN_POINT ( 'NONE',  ( 2.899999999999944844, 12.50000000000000000, 4.957854068765711553 ) ) ;
#96383=CONICAL_SURFACE ( 'NONE', #111044, 0.09999999999999982514, 0.003490658503988666988 ) ;
#96384=CONICAL_SURFACE ( 'NONE', #86005, 0.1000000000000000472, 0.003490658503988666988 ) ;
#96385=VERTEX_POINT ( 'NONE', #79240 ) ;
#96386=DIRECTION ( 'NONE',  ( 0.000000000000000000, 1.000000000000000000, 0.000000000000000000 ) ) ;
#96387=ORIENTED_EDGE ( 'NONE', *, *, #104305, .T. ) ;
#96388=CARTESIAN_POINT ( 'NONE',  ( -8.300000000000011369, 2.500000000000000000, -4.230127018922201998 ) ) ;
#96389=DIRECTION ( 'NONE',  ( 0.000000000000000000, 1.000000000000000000, 0.000000000000000000 ) ) ;
#96390=EDGE_CURVE ( 'NONE', #83631, #49637, #58952, .T. ) ;
#96391=CIRCLE ( 'NONE', #75471, 0.1000000000000000472 ) ;
#96392=DIRECTION ( 'NONE',  ( 0.000000000000000000, 0.000000000000000000, 1.000000000000000000 ) ) ;
#96393=EDGE_LOOP ( 'NONE', ( #42926, #9817, #57971, #11249 ) ) ;
#96394=EDGE_CURVE ( 'NONE', #82278, #49864, #38685, .T. ) ;
#96395=DIRECTION ( 'NONE',  ( -0.000000000000000000, -1.000000000000000000, -0.000000000000000000 ) ) ;
#96396=EDGE_CURVE ( 'NONE', #48604, #28288, #9647, .T. ) ;
#96397=DIRECTION ( 'NONE',  ( 0.000000000000000000, 0.000000000000000000, -1.000000000000000000 ) ) ;
#96398=VECTOR ( 'NONE', #114149, 1000.000000000000000 ) ;
#96399=AXIS2_PLACEMENT_3D ( 'NONE', #26635, #66546, #129376 ) ;
#96400=ORIENTED_EDGE ( 'NONE', *, *, #127851, .T. ) ;
#96401=VERTEX_POINT ( 'NONE', #18364 ) ;
#96402=FACE_OUTER_BOUND ( 'NONE', #74722, .T. ) ;
#96403=EDGE_LOOP ( 'NONE', ( #113854, #40812 ) ) ;
#96405=CARTESIAN_POINT ( 'NONE',  ( -3.950000000000026379, 2.500000000000000000, 2.611473670974873151 ) ) ;
#96406=EDGE_LOOP ( 'NONE', ( #101153, #34998 ) ) ;
#96407=VERTEX_POINT ( 'NONE', #60874 ) ;
#96408=CARTESIAN_POINT ( 'NONE',  ( -8.100000000000010303, 2.500000000000000000, 4.576537180435972019 ) ) ;
#96409=FACE_OUTER_BOUND ( 'NONE', #107286, .T. ) ;
#96410=ORIENTED_EDGE ( 'NONE', *, *, #109397, .T. ) ;
#96411=DIRECTION ( 'NONE',  ( 0.000000000000000000, -0.000000000000000000, 1.000000000000000000 ) ) ;
#96412=CARTESIAN_POINT ( 'NONE',  ( 14.54999999999989235, 2.500000000000000000, -2.265063509461101798 ) ) ;
#96413=AXIS2_PLACEMENT_3D ( 'NONE', #34713, #6472, #87639 ) ;
#96414=CARTESIAN_POINT ( 'NONE',  ( -11.44999999999999929, 12.50000000000000000, -6.083687093685485436 ) ) ;
#96416=AXIS2_PLACEMENT_3D ( 'NONE', #119859, #84281, #34568 ) ;
#96417=AXIS2_PLACEMENT_3D ( 'NONE', #89258, #27747, #69611 ) ;
#96418=DIRECTION ( 'NONE',  ( 0.000000000000000000, 0.000000000000000000, 1.000000000000000000 ) ) ;
#96420=CIRCLE ( 'NONE', #40022, 0.09999999999999982514 ) ;
#96421=ORIENTED_EDGE ( 'NONE', *, *, #37870, .F. ) ;
#96422=CONICAL_SURFACE ( 'NONE', #40024, 0.1000000000000000056, 0.003490658503988666988 ) ;
#96423=ORIENTED_EDGE ( 'NONE', *, *, #119114, .T. ) ;
#96424=ORIENTED_EDGE ( 'NONE', *, *, #25300, .F. ) ;
#96425=VERTEX_POINT ( 'NONE', #98213 ) ;
#96426=FACE_OUTER_BOUND ( 'NONE', #89076, .T. ) ;
#96427=CARTESIAN_POINT ( 'NONE',  ( 2.499999999999983569, 12.50000000000000000, -4.265033745738164406 ) ) ;
#96428=AXIS2_PLACEMENT_3D ( 'NONE', #89247, #39537, #79444 ) ;
#96429=DIRECTION ( 'NONE',  ( 0.000000000000000000, -0.9999939076577903929, 0.003490651415223739937 ) ) ;
#96430=EDGE_LOOP ( 'NONE', ( #9131, #65056 ) ) ;
#96431=FACE_BOUND ( 'NONE', #66356, .T. ) ;
#96432=ADVANCED_FACE ( 'NONE', ( #120444 ), #659, .T. ) ;
#96433=DIRECTION ( 'NONE',  ( -0.000000000000000000, -1.000000000000000000, -0.000000000000000000 ) ) ;
#96434=LINE ( 'NONE', #37544, #16640 ) ;
#96436=DIRECTION ( 'NONE',  ( -4.274815082592931898E-19, -0.9999939076577903929, -0.003490651415223739937 ) ) ;
#96437=DIRECTION ( 'NONE',  ( 0.000000000000000000, 0.000000000000000000, 1.000000000000000000 ) ) ;
#96438=EDGE_CURVE ( 'NONE', #115346, #41126, #78605, .T. ) ;
#96439=PLANE ( 'NONE',  #24189 ) ;
#96440=DIRECTION ( 'NONE',  ( -0.000000000000000000, -1.000000000000000000, -0.000000000000000000 ) ) ;
#96441=DIRECTION ( 'NONE',  ( 0.000000000000000000, 0.000000000000000000, 1.000000000000000000 ) ) ;
#96442=FACE_OUTER_BOUND ( 'NONE', #117769, .T. ) ;
#96443=FACE_OUTER_BOUND ( 'NONE', #31674, .T. ) ;
#96444=CARTESIAN_POINT ( 'NONE',  ( 9.349999999999919709, 12.50000000000000000, -6.213873640053564351 ) ) ;
#96445=EDGE_CURVE ( 'NONE', #22282, #128788, #5428, .T. ) ;
#96446=EDGE_LOOP ( 'NONE', ( #12271, #42372, #101404, #126333 ) ) ;
#96447=ORIENTED_EDGE ( 'NONE', *, *, #129283, .F. ) ;
#96448=ORIENTED_EDGE ( 'NONE', *, *, #95877, .F. ) ;
#96449=ORIENTED_EDGE ( 'NONE', *, *, #97197, .F. ) ;
#96450=DIRECTION ( 'NONE',  ( 0.000000000000000000, 0.000000000000000000, 1.000000000000000000 ) ) ;
#96451=DIRECTION ( 'NONE',  ( -0.000000000000000000, 1.000000000000000000, -0.000000000000000000 ) ) ;
#96452=ORIENTED_EDGE ( 'NONE', *, *, #7725, .F. ) ;
#96453=EDGE_LOOP ( 'NONE', ( #76210, #119984 ) ) ;
#96454=ORIENTED_EDGE ( 'NONE', *, *, #56126, .T. ) ;
#96455=FACE_OUTER_BOUND ( 'NONE', #94198, .T. ) ;
#96456=CIRCLE ( 'NONE', #65142, 0.06509327318403745899 ) ;
#96457=CIRCLE ( 'NONE', #121493, 0.1000000000000002554 ) ;
#96458=CARTESIAN_POINT ( 'NONE',  ( 4.913542845177470753, -1.500000000000381473, 9.942462991075531775 ) ) ;
#96459=DIRECTION ( 'NONE',  ( -0.000000000000000000, 1.000000000000000000, -0.000000000000000000 ) ) ;
#96460=DIRECTION ( 'NONE',  ( -0.000000000000000000, 1.000000000000000000, -0.000000000000000000 ) ) ;
#96461=DIRECTION ( 'NONE',  ( 0.000000000000000000, -0.000000000000000000, 1.000000000000000000 ) ) ;
#96462=EDGE_LOOP ( 'NONE', ( #1364, #31192, #113105, #64425 ) ) ;
#96463=CONICAL_SURFACE ( 'NONE', #42112, 0.1000000000000000056, 0.003490658503988666988 ) ;
#96464=ORIENTED_EDGE ( 'NONE', *, *, #38869, .F. ) ;
#96465=EDGE_LOOP ( 'NONE', ( #76342, #54284 ) ) ;
#96466=AXIS2_PLACEMENT_3D ( 'NONE', #41019, #21347, #51470 ) ;
#96467=ORIENTED_EDGE ( 'NONE', *, *, #92572, .T. ) ;
#96468=DIRECTION ( 'NONE',  ( -4.274815082592931898E-19, -0.9999939076577903929, -0.003490651415223739937 ) ) ;
#96469=ORIENTED_EDGE ( 'NONE', *, *, #127682, .F. ) ;
#96470=ORIENTED_EDGE ( 'NONE', *, *, #16942, .F. ) ;
#96472=CARTESIAN_POINT ( 'NONE',  ( -9.999999999999969802, 2.500000000000000000, 0.09999999999999772959 ) ) ;
#96473=CIRCLE ( 'NONE', #40063, 0.06509327318403745899 ) ;
#96474=CARTESIAN_POINT ( 'NONE',  ( 8.349999999999919709, 2.500000000000000000, -1.472243186433550122 ) ) ;
#96475=CARTESIAN_POINT ( 'NONE',  ( -12.89999999999999147, 2.500000000000000000, 5.022947341949748790 ) ) ;
#96476=EDGE_CURVE ( 'NONE', #71888, #22161, #9196, .T. ) ;
#96477=FACE_OUTER_BOUND ( 'NONE', #1331, .T. ) ;
#96478=AXIS2_PLACEMENT_3D ( 'NONE', #73042, #72409, #60659 ) ;
#96479=CARTESIAN_POINT ( 'NONE',  ( 9.799999999999918998, 12.50000000000000000, -0.2813168883297408329 ) ) ;
#96480=ORIENTED_EDGE ( 'NONE', *, *, #40688, .T. ) ;
#96481=DIRECTION ( 'NONE',  ( 0.000000000000000000, 0.000000000000000000, 1.000000000000000000 ) ) ;
#96482=VERTEX_POINT ( 'NONE', #69396 ) ;
#96483=DIRECTION ( 'NONE',  ( -0.000000000000000000, 1.000000000000000000, -0.000000000000000000 ) ) ;
#96484=ORIENTED_EDGE ( 'NONE', *, *, #42626, .F. ) ;
#96485=DIRECTION ( 'NONE',  ( 0.000000000000000000, 0.000000000000000000, -1.000000000000000000 ) ) ;
#96486=VECTOR ( 'NONE', #77440, 1000.000000000000000 ) ;
#96487=AXIS2_PLACEMENT_3D ( 'NONE', #110346, #21991, #79602 ) ;
#96488=FACE_OUTER_BOUND ( 'NONE', #47311, .T. ) ;
#96489=VERTEX_POINT ( 'NONE', #119794 ) ;
#96490=DIRECTION ( 'NONE',  ( 0.000000000000000000, 0.000000000000000000, 1.000000000000000000 ) ) ;
#96491=ADVANCED_FACE ( 'NONE', ( #94203 ), #45166, .T. ) ;
#96492=CARTESIAN_POINT ( 'NONE',  ( -11.25000000000000178, 12.50000000000000000, -1.472243186433546125 ) ) ;
#96493=ORIENTED_EDGE ( 'NONE', *, *, #87411, .F. ) ;
#96494=DIRECTION ( 'NONE',  ( 0.000000000000000000, 0.000000000000000000, -1.000000000000000000 ) ) ;
#96495=ORIENTED_EDGE ( 'NONE', *, *, #2203, .F. ) ;
#96496=EDGE_CURVE ( 'NONE', #123090, #126709, #52995, .T. ) ;
#96497=VERTEX_POINT ( 'NONE', #41256 ) ;
#96498=DIRECTION ( 'NONE',  ( 0.000000000000000000, 0.000000000000000000, -1.000000000000000000 ) ) ;
#96499=DIRECTION ( 'NONE',  ( 0.000000000000000000, 0.000000000000000000, 1.000000000000000000 ) ) ;
#96501=DIRECTION ( 'NONE',  ( 0.000000000000000000, 0.000000000000000000, 1.000000000000000000 ) ) ;
#96502=CARTESIAN_POINT ( 'NONE',  ( 4.599999999999939249, 12.50000000000000000, -3.702399969078687292 ) ) ;
#96503=CARTESIAN_POINT ( 'NONE',  ( 14.54999999999989235, 2.500000000000000000, -2.265063509461101798 ) ) ;
#96504=AXIS2_PLACEMENT_3D ( 'NONE', #31396, #71966, #81756 ) ;
#96505=VECTOR ( 'NONE', #123239, 1000.000000000000000 ) ;
#96506=ORIENTED_EDGE ( 'NONE', *, *, #11407, .F. ) ;
#96507=FACE_OUTER_BOUND ( 'NONE', #131, .T. ) ;
#96508=AXIS2_PLACEMENT_3D ( 'NONE', #40563, #79813, #60827 ) ;
#96509=AXIS2_PLACEMENT_3D ( 'NONE', #106772, #103080, #13399 ) ;
#96510=ADVANCED_FACE ( 'NONE', ( #54279 ), #103652, .T. ) ;
#96511=VERTEX_POINT ( 'NONE', #104029 ) ;
#96512=CIRCLE ( 'NONE', #54759, 0.06509327318403745899 ) ;
#96513=CONICAL_SURFACE ( 'NONE', #63088, 0.1000000000000000472, 0.003490658503988666988 ) ;
#96514=DIRECTION ( 'NONE',  ( 0.000000000000000000, 0.000000000000000000, 1.000000000000000000 ) ) ;
#96515=FACE_OUTER_BOUND ( 'NONE', #51848, .T. ) ;
#96516=LINE ( 'NONE', #77535, #69452 ) ;
#96517=DIRECTION ( 'NONE',  ( 0.000000000000000000, 0.000000000000000000, 1.000000000000000000 ) ) ;
#96518=DIRECTION ( 'NONE',  ( 0.000000000000000000, 1.000000000000000000, 0.000000000000000000 ) ) ;
#96519=ORIENTED_EDGE ( 'NONE', *, *, #25895, .F. ) ;
#96520=EDGE_CURVE ( 'NONE', #63624, #119823, #1238, .T. ) ;
#96521=DIRECTION ( 'NONE',  ( 0.000000000000000000, 1.000000000000000000, 0.000000000000000000 ) ) ;
#96522=DIRECTION ( 'NONE',  ( 0.000000000000000000, 0.000000000000000000, -1.000000000000000000 ) ) ;
#96523=ADVANCED_FACE ( 'NONE', ( #63462 ), #103384, .T. ) ;
#96524=EDGE_CURVE ( 'NONE', #20444, #3575, #33372, .T. ) ;
#96525=EDGE_CURVE ( 'NONE', #20333, #10004, #7490, .T. ) ;
#96526=EDGE_CURVE ( 'NONE', #114323, #101653, #22264, .T. ) ;
#96527=VERTEX_POINT ( 'NONE', #121722 ) ;
#96528=DIRECTION ( 'NONE',  ( -0.000000000000000000, 1.000000000000000000, -0.000000000000000000 ) ) ;
#96529=ORIENTED_EDGE ( 'NONE', *, *, #41220, .F. ) ;
#96530=ORIENTED_EDGE ( 'NONE', *, *, #50270, .F. ) ;
#96531=CARTESIAN_POINT ( 'NONE',  ( 9.149999999999916866, 2.500000000000000000, 7.088010851410848190 ) ) ;
#96532=EDGE_CURVE ( 'NONE', #69316, #51138, #22189, .T. ) ;
#96534=VERTEX_POINT ( 'NONE', #23522 ) ;
#96535=CARTESIAN_POINT ( 'NONE',  ( -6.700000000000016165, 2.500000000000000000, 4.330127018922196314 ) ) ;
#96536=FACE_OUTER_BOUND ( 'NONE', #123683, .T. ) ;
#96537=FACE_OUTER_BOUND ( 'NONE', #45942, .T. ) ;
#96538=CONICAL_SURFACE ( 'NONE', #107005, 0.09999999999999982514, 0.003490658503988666988 ) ;
#96539=ORIENTED_EDGE ( 'NONE', *, *, #107130, .T. ) ;
#96540=VECTOR ( 'NONE', #65601, 1000.000000000000000 ) ;
#96541=EDGE_CURVE ( 'NONE', #62955, #67958, #102715, .T. ) ;
#96542=FACE_BOUND ( 'NONE', #95581, .T. ) ;
#96543=EDGE_CURVE ( 'NONE', #86820, #63617, #93191, .T. ) ;
#96544=DIRECTION ( 'NONE',  ( -0.000000000000000000, 1.000000000000000000, -0.000000000000000000 ) ) ;
#96545=ORIENTED_EDGE ( 'NONE', *, *, #30411, .T. ) ;
#96546=CARTESIAN_POINT ( 'NONE',  ( 4.999999999999936939, 2.500000000000000000, -0.6928203230275541413 ) ) ;
#96547=DIRECTION ( 'NONE',  ( 0.000000000000000000, 1.000000000000000000, 0.000000000000000000 ) ) ;
#96548=AXIS2_PLACEMENT_3D ( 'NONE', #48268, #97368, #77712 ) ;
#96549=ADVANCED_FACE ( 'NONE', ( #111240 ), #13741, .T. ) ;
#96550=ADVANCED_FACE ( 'NONE', ( #24177 ), #30510, .T. ) ;
#96551=ORIENTED_EDGE ( 'NONE', *, *, #69446, .F. ) ;
#96552=AXIS2_PLACEMENT_3D ( 'NONE', #60612, #62539, #40322 ) ;
#96553=CIRCLE ( 'NONE', #17117, 0.06509327318403745899 ) ;
#96554=EDGE_LOOP ( 'NONE', ( #101295, #31553, #114951, #118471 ) ) ;
#96555=ORIENTED_EDGE ( 'NONE', *, *, #25797, .F. ) ;
#96556=DIRECTION ( 'NONE',  ( 0.000000000000000000, 0.000000000000000000, -1.000000000000000000 ) ) ;
#96557=LINE ( 'NONE', #58597, #60367 ) ;
#96558=DIRECTION ( 'NONE',  ( 0.000000000000000000, 0.000000000000000000, -1.000000000000000000 ) ) ;
#96559=FACE_BOUND ( 'NONE', #82922, .T. ) ;
#96560=ORIENTED_EDGE ( 'NONE', *, *, #18074, .F. ) ;
#96561=DIRECTION ( 'NONE',  ( 0.000000000000000000, 0.000000000000000000, 1.000000000000000000 ) ) ;
#96562=CARTESIAN_POINT ( 'NONE',  ( -11.89999999999999680, 12.50000000000000000, -4.676537180435976104 ) ) ;
#96563=CIRCLE ( 'NONE', #33891, 0.09999999999999982514 ) ;
#96564=CONICAL_SURFACE ( 'NONE', #77787, 0.1000000000000002554, 0.003490658503988666988 ) ;
#96565=FACE_OUTER_BOUND ( 'NONE', #125471, .T. ) ;
#96566=CIRCLE ( 'NONE', #54811, 0.1000000000000000472 ) ;
#96567=VECTOR ( 'NONE', #96320, 1000.000000000000000 ) ;
#96568=CONICAL_SURFACE ( 'NONE', #31844, 0.09999999999999982514, 0.003490658503988666988 ) ;
#96569=DIRECTION ( 'NONE',  ( 0.000000000000000000, 0.000000000000000000, 1.000000000000000000 ) ) ;
#96570=DIRECTION ( 'NONE',  ( 0.000000000000000000, 1.000000000000000000, 0.000000000000000000 ) ) ;
#96571=CARTESIAN_POINT ( 'NONE',  ( -8.350000000000012079, 12.50000000000000000, 2.922977105672686982 ) ) ;
#96572=CIRCLE ( 'NONE', #104986, 0.1000000000000002554 ) ;
#96573=DIRECTION ( 'NONE',  ( 0.000000000000000000, -0.9999939076577903929, 0.003490651415223739937 ) ) ;
#96574=ORIENTED_EDGE ( 'NONE', *, *, #20183, .F. ) ;
#96575=CIRCLE ( 'NONE', #27526, 0.06509327318403745899 ) ;
#96576=ORIENTED_EDGE ( 'NONE', *, *, #9099, .F. ) ;
#96577=ORIENTED_EDGE ( 'NONE', *, *, #115973, .F. ) ;
#96578=ORIENTED_EDGE ( 'NONE', *, *, #79518, .T. ) ;
#96579=EDGE_LOOP ( 'NONE', ( #74792, #45596 ) ) ;
#96580=DIRECTION ( 'NONE',  ( -0.000000000000000000, -1.000000000000000000, -0.000000000000000000 ) ) ;
#96581=PLANE ( 'NONE',  #96857 ) ;
#96582=EDGE_LOOP ( 'NONE', ( #5822, #112205 ) ) ;
#96583=FACE_BOUND ( 'NONE', #841, .T. ) ;
#96584=CARTESIAN_POINT ( 'NONE',  ( 11.64999999999990798, 2.500000000000000000, -1.372243186433550033 ) ) ;
#96585=ADVANCED_FACE ( 'NONE', ( #51712 ), #41899, .T. ) ;
#96586=CARTESIAN_POINT ( 'NONE',  ( 3.349999999999941913, 2.500000000000000000, 5.702370205355745014 ) ) ;
#96587=EDGE_CURVE ( 'NONE', #86863, #21611, #26380, .T. ) ;
#96588=DIRECTION ( 'NONE',  ( 0.000000000000000000, -0.000000000000000000, 1.000000000000000000 ) ) ;
#96589=FACE_OUTER_BOUND ( 'NONE', #67080, .T. ) ;
#96590=DIRECTION ( 'NONE',  ( 0.000000000000000000, 0.000000000000000000, 1.000000000000000000 ) ) ;
#96591=EDGE_LOOP ( 'NONE', ( #111916, #48403, #111101, #96825 ) ) ;
#96592=DIRECTION ( 'NONE',  ( 0.000000000000000000, 0.000000000000000000, 1.000000000000000000 ) ) ;
#96593=ORIENTED_EDGE ( 'NONE', *, *, #82404, .F. ) ;
#96594=VERTEX_POINT ( 'NONE', #2578 ) ;
#96595=VERTEX_POINT ( 'NONE', #82468 ) ;
#96596=AXIS2_PLACEMENT_3D ( 'NONE', #46023, #15234, #76115 ) ;
#96598=CIRCLE ( 'NONE', #123788, 0.09999999999999982514 ) ;
#96599=CARTESIAN_POINT ( 'NONE',  ( 4.849235612580145016, 2.499999999999999556, 8.943930330244967308 ) ) ;
#96600=DIRECTION ( 'NONE',  ( 0.000000000000000000, -0.000000000000000000, 1.000000000000000000 ) ) ;
#96601=ORIENTED_EDGE ( 'NONE', *, *, #18703, .T. ) ;
#96602=CARTESIAN_POINT ( 'NONE',  ( 7.306656945318586338, 1.500000000000379918, -9.704971168320692954 ) ) ;
#96603=CARTESIAN_POINT ( 'NONE',  ( 12.09999999999990195, 2.500000000000000000, -0.6928203230275541413 ) ) ;
#96605=CIRCLE ( 'NONE', #109127, 0.06509327318403745899 ) ;
#96606=DIRECTION ( 'NONE',  ( 0.000000000000000000, 1.000000000000000000, 0.000000000000000000 ) ) ;
#96608=DIRECTION ( 'NONE',  ( -0.000000000000000000, -1.000000000000000000, -0.000000000000000000 ) ) ;
#96609=DIRECTION ( 'NONE',  ( -0.000000000000000000, -1.000000000000000000, -0.000000000000000000 ) ) ;
#96610=CONICAL_SURFACE ( 'NONE', #100820, 0.1000000000000000472, 0.003490658503988666988 ) ;
#96611=AXIS2_PLACEMENT_3D ( 'NONE', #54944, #56232, #86986 ) ;
#96612=CARTESIAN_POINT ( 'NONE',  ( -10.84999999999999964, 2.500000000000000000, 1.572243186433545548 ) ) ;
#96613=VERTEX_POINT ( 'NONE', #112567 ) ;
#96614=DIRECTION ( 'NONE',  ( -0.000000000000000000, 1.000000000000000000, -0.000000000000000000 ) ) ;
#96615=AXIS2_PLACEMENT_3D ( 'NONE', #46282, #6981, #95394 ) ;
#96616=ORIENTED_EDGE ( 'NONE', *, *, #78766, .F. ) ;
#96617=ORIENTED_EDGE ( 'NONE', *, *, #71054, .F. ) ;
#96618=DIRECTION ( 'NONE',  ( -0.000000000000000000, -1.000000000000000000, -0.000000000000000000 ) ) ;
#96619=DIRECTION ( 'NONE',  ( -4.274815082592931898E-19, -0.9999939076577903929, -0.003490651415223739937 ) ) ;
#96620=FACE_OUTER_BOUND ( 'NONE', #123745, .T. ) ;
#96621=EDGE_LOOP ( 'NONE', ( #118682, #5345 ) ) ;
#96622=VERTEX_POINT ( 'NONE', #22899 ) ;
#96623=ADVANCED_FACE ( 'NONE', ( #37232 ), #17959, .T. ) ;
#96624=DIRECTION ( 'NONE',  ( 0.000000000000000000, 0.000000000000000000, -1.000000000000000000 ) ) ;
#96625=CARTESIAN_POINT ( 'NONE',  ( -7.500000000000011546, 2.500000000000000000, 3.637306695894644726 ) ) ;
#96626=CARTESIAN_POINT ( 'NONE',  ( 8.749999999999957367, 12.50000000000000000, -6.495190528383302464 ) ) ;
#96627=ORIENTED_EDGE ( 'NONE', *, *, #122287, .F. ) ;
#96628=ORIENTED_EDGE ( 'NONE', *, *, #113346, .F. ) ;
#96629=DIRECTION ( 'NONE',  ( -4.274815082592931898E-19, -0.9999939076577903929, -0.003490651415223739937 ) ) ;
#96630=VECTOR ( 'NONE', #258, 1000.000000000000000 ) ;
#96631=ORIENTED_EDGE ( 'NONE', *, *, #72780, .F. ) ;
#96632=DIRECTION ( 'NONE',  ( -0.000000000000000000, 1.000000000000000000, -0.000000000000000000 ) ) ;
#96633=FACE_OUTER_BOUND ( 'NONE', #43336, .T. ) ;
#96634=VERTEX_POINT ( 'NONE', #16261 ) ;
#96635=CARTESIAN_POINT ( 'NONE',  ( 8.149999999999923972, 12.50000000000000000, 1.753560074763284016 ) ) ;
#96636=CARTESIAN_POINT ( 'NONE',  ( 11.04999999999991012, 2.500000000000000000, 6.941600689897073018 ) ) ;
#96637=DIRECTION ( 'NONE',  ( 0.000000000000000000, 0.000000000000000000, 1.000000000000000000 ) ) ;
#96638=ADVANCED_FACE ( 'NONE', ( #75840 ), #99544, .T. ) ;
#96639=EDGE_CURVE ( 'NONE', #11311, #37370, #116242, .T. ) ;
#96640=CARTESIAN_POINT ( 'NONE',  ( 8.749999999999957367, 2.500000000000000000, 2.165063509461097713 ) ) ;
#96641=CIRCLE ( 'NONE', #105055, 0.06509327318403745899 ) ;
#96642=ORIENTED_EDGE ( 'NONE', *, *, #117601, .F. ) ;
#96643=VECTOR ( 'NONE', #68966, 1000.000000000000000 ) ;
#96644=CONICAL_SURFACE ( 'NONE', #105058, 0.1000000000000002554, 0.003490658503988666988 ) ;
#96645=CARTESIAN_POINT ( 'NONE',  ( -11.64999999999999680, 2.500000000000000000, 1.572243186433545548 ) ) ;
#96646=CIRCLE ( 'NONE', #63217, 0.06509327318403745899 ) ;
#96648=ORIENTED_EDGE ( 'NONE', *, *, #113973, .T. ) ;
#96649=VERTEX_POINT ( 'NONE', #47048 ) ;
#96650=EDGE_CURVE ( 'NONE', #78527, #68389, #74563, .T. ) ;
#96652=CARTESIAN_POINT ( 'NONE',  ( -10.40000000000000213, 2.500000000000000000, 3.537306695894645081 ) ) ;
#96653=CARTESIAN_POINT ( 'NONE',  ( -7.950000000000009059, 2.500000000000000000, 6.595190528383296780 ) ) ;
#96655=VECTOR ( 'NONE', #75310, 1000.000000000000000 ) ;
#96656=DIRECTION ( 'NONE',  ( 0.000000000000000000, -0.9999939076577903929, 0.003490651415223739937 ) ) ;
#96657=DIRECTION ( 'NONE',  ( 0.000000000000000000, 1.000000000000000000, 0.000000000000000000 ) ) ;
#96658=CIRCLE ( 'NONE', #123854, 0.09999999999999982514 ) ;
#96659=CARTESIAN_POINT ( 'NONE',  ( 16.88398418147296809, 2.500000000000000000, -4.430584152985972857 ) ) ;
#96660=CONICAL_SURFACE ( 'NONE', #98721, 0.09999999999999999167, 0.003490658503988666988 ) ;
#96661=CARTESIAN_POINT ( 'NONE',  ( 1.649999999999951505, 2.500000000000000000, 2.857883832488649301 ) ) ;
#96662=CIRCLE ( 'NONE', #36047, 0.06509327318403741736 ) ;
#96663=VECTOR ( 'NONE', #114494, 1000.000000000000000 ) ;
#96664=PLANE ( 'NONE',  #104826 ) ;
#96665=AXIS2_PLACEMENT_3D ( 'NONE', #64074, #33350, #104003 ) ;
#96666=CARTESIAN_POINT ( 'NONE',  ( 3.949999999999941558, 12.50000000000000000, -1.753560074763288679 ) ) ;
#96667=CONICAL_SURFACE ( 'NONE', #79963, 0.1000000000000000056, 0.003490658503988666988 ) ;
#96668=ORIENTED_EDGE ( 'NONE', *, *, #81354, .T. ) ;
#96669=DIRECTION ( 'NONE',  ( 0.000000000000000000, 0.000000000000000000, 1.000000000000000000 ) ) ;
#96670=EDGE_LOOP ( 'NONE', ( #77129, #9859 ) ) ;
#96671=DIRECTION ( 'NONE',  ( -0.000000000000000000, -1.000000000000000000, -0.000000000000000000 ) ) ;
#96672=FACE_OUTER_BOUND ( 'NONE', #56202, .T. ) ;
#96673=CARTESIAN_POINT ( 'NONE',  ( -10.60000000000000142, 2.500000000000000000, 4.676537180435972552 ) ) ;
#96674=ORIENTED_EDGE ( 'NONE', *, *, #116340, .F. ) ;
#96675=CARTESIAN_POINT ( 'NONE',  ( -12.29999999999999538, 12.50000000000000000, -0.2813168883297367806 ) ) ;
#96676=ADVANCED_FACE ( 'NONE', ( #85667 ), #77143, .T. ) ;
#96677=DIRECTION ( 'NONE',  ( -0.000000000000000000, 1.000000000000000000, -0.000000000000000000 ) ) ;
#96678=CARTESIAN_POINT ( 'NONE',  ( -6.650000000000015454, 2.500000000000000000, 2.957883832488649389 ) ) ;
#96679=ORIENTED_EDGE ( 'NONE', *, *, #68461, .F. ) ;
#96680=AXIS2_PLACEMENT_3D ( 'NONE', #70769, #2652, #42619 ) ;
#96681=EDGE_CURVE ( 'NONE', #8138, #79642, #40973, .T. ) ;
#96682=EDGE_CURVE ( 'NONE', #63281, #8031, #112056, .T. ) ;
#96683=LINE ( 'NONE', #14267, #45843 ) ;
#96684=ORIENTED_EDGE ( 'NONE', *, *, #14699, .T. ) ;
#96685=ORIENTED_EDGE ( 'NONE', *, *, #9125, .F. ) ;
#96686=ORIENTED_EDGE ( 'NONE', *, *, #117217, .F. ) ;
#96687=VECTOR ( 'NONE', #119435, 1000.000000000000000 ) ;
#96688=ORIENTED_EDGE ( 'NONE', *, *, #12449, .F. ) ;
#96689=DIRECTION ( 'NONE',  ( 0.000000000000000000, 1.000000000000000000, 0.000000000000000000 ) ) ;
#96690=VECTOR ( 'NONE', #83122, 1000.000000000000000 ) ;
#96691=ADVANCED_FACE ( 'NONE', ( #115102 ), #84856, .T. ) ;
#96692=CIRCLE ( 'NONE', #42341, 0.06509327318403741736 ) ;
#96693=EDGE_CURVE ( 'NONE', #126609, #128794, #105317, .T. ) ;
#96694=EDGE_CURVE ( 'NONE', #110810, #125867, #55571, .T. ) ;
#96695=DIRECTION ( 'NONE',  ( 0.9974916312695814025, 0.05217691604167131597, 0.04783319955355550684 ) ) ;
#96696=DIRECTION ( 'NONE',  ( 0.000000000000000000, 1.000000000000000000, 0.000000000000000000 ) ) ;
#96697=CARTESIAN_POINT ( 'NONE',  ( -14.99999999999998401, 2.500000000000000000, 0.7928203230275517877 ) ) ;
#96698=AXIS2_PLACEMENT_3D ( 'NONE', #3299, #43243, #119845 ) ;
#96699=ORIENTED_EDGE ( 'NONE', *, *, #66247, .T. ) ;
#96700=AXIS2_PLACEMENT_3D ( 'NONE', #71923, #111836, #102645 ) ;
#96701=AXIS2_PLACEMENT_3D ( 'NONE', #122140, #72397, #13447 ) ;
#96702=EDGE_CURVE ( 'NONE', #97511, #109623, #28441, .T. ) ;
#96703=CARTESIAN_POINT ( 'NONE',  ( -6.450000000000014388, 12.50000000000000000, 6.213873640053559022 ) ) ;
#96704=CIRCLE ( 'NONE', #90438, 0.1000000000000000472 ) ;
#96705=VERTEX_POINT ( 'NONE', #26754 ) ;
#96706=CARTESIAN_POINT ( 'NONE',  ( 59.88499455115334769, -2.860410828890750157, -5.641292085239668630 ) ) ;
#96707=DIRECTION ( 'NONE',  ( 0.000000000000000000, 0.000000000000000000, 1.000000000000000000 ) ) ;
#96708=VECTOR ( 'NONE', #118155, 1000.000000000000000 ) ;
#96709=LINE ( 'NONE', #124900, #92322 ) ;
#96710=CIRCLE ( 'NONE', #61227, 0.1000000000000002554 ) ;
#96711=FACE_OUTER_BOUND ( 'NONE', #104850, .T. ) ;
#96712=EDGE_CURVE ( 'NONE', #27192, #17818, #96131, .T. ) ;
#96713=AXIS2_PLACEMENT_3D ( 'NONE', #99273, #48887, #60006 ) ;
#96714=ORIENTED_EDGE ( 'NONE', *, *, #65356, .F. ) ;
#96715=EDGE_LOOP ( 'NONE', ( #26177, #53974, #54134, #78124 ) ) ;
#96716=ORIENTED_EDGE ( 'NONE', *, *, #52377, .F. ) ;
#96717=ORIENTED_EDGE ( 'NONE', *, *, #35258, .F. ) ;
#96718=DIRECTION ( 'NONE',  ( 0.000000000000000000, 0.000000000000000000, 1.000000000000000000 ) ) ;
#96719=CARTESIAN_POINT ( 'NONE',  ( 87.50000000000001421, 3.975350567648425759, 6.360562287258741065 ) ) ;
#96720=DIRECTION ( 'NONE',  ( -4.274815082592931898E-19, -0.9999939076577903929, -0.003490651415223739937 ) ) ;
#96721=FACE_BOUND ( 'NONE', #60859, .T. ) ;
#96723=PLANE ( 'NONE',  #100969 ) ;
#96724=FACE_OUTER_BOUND ( 'NONE', #55831, .T. ) ;
#96725=CARTESIAN_POINT ( 'NONE',  ( -3.950000000000024603, 12.50000000000000000, -2.576566944158915184 ) ) ;
#96727=DIRECTION ( 'NONE',  ( 0.000000000000000000, 0.000000000000000000, 1.000000000000000000 ) ) ;
#96728=DIRECTION ( 'NONE',  ( 0.000000000000000000, 1.000000000000000000, 0.000000000000000000 ) ) ;
#96729=AXIS2_PLACEMENT_3D ( 'NONE', #109258, #55818, #116021 ) ;
#96730=AXIS2_PLACEMENT_3D ( 'NONE', #51380, #10754, #120740 ) ;
#96731=AXIS2_PLACEMENT_3D ( 'NONE', #36082, #84533, #36740 ) ;
#96732=DIRECTION ( 'NONE',  ( 0.000000000000000000, 0.000000000000000000, 1.000000000000000000 ) ) ;
#96733=EDGE_LOOP ( 'NONE', ( #60809, #67217 ) ) ;
#96734=VERTEX_POINT ( 'NONE', #14961 ) ;
#96735=ORIENTED_EDGE ( 'NONE', *, *, #86370, .T. ) ;
#96736=ORIENTED_EDGE ( 'NONE', *, *, #76289, .F. ) ;
#96737=DIRECTION ( 'NONE',  ( 0.000000000000000000, 1.000000000000000000, 0.000000000000000000 ) ) ;
#96738=FACE_BOUND ( 'NONE', #127095, .T. ) ;
#96739=CONICAL_SURFACE ( 'NONE', #34070, 0.1000000000000002554, 0.003490658503988666988 ) ;
#96740=DIRECTION ( 'NONE',  ( 0.000000000000000000, 0.000000000000000000, -1.000000000000000000 ) ) ;
#96741=CARTESIAN_POINT ( 'NONE',  ( 7.949999999999922018, 2.500000000000000000, -2.265063509461101798 ) ) ;
#96742=CONICAL_SURFACE ( 'NONE', #86276, 0.09999999999999982514, 0.003490658503988666988 ) ;
#96743=ADVANCED_FACE ( 'NONE', ( #26115 ), #105790, .T. ) ;
#96744=ORIENTED_EDGE ( 'NONE', *, *, #112240, .T. ) ;
#96745=CARTESIAN_POINT ( 'NONE',  ( -3.950000000000026379, 12.50000000000000000, -1.753560074763288679 ) ) ;
#96747=EDGE_LOOP ( 'NONE', ( #126656, #5401 ) ) ;
#96749=CARTESIAN_POINT ( 'NONE',  ( 19.95908882845296617, 2.629614671951221005, -2.273431397254392916 ) ) ;
#96750=AXIS2_PLACEMENT_3D ( 'NONE', #635, #100761, #58929 ) ;
#96751=EDGE_CURVE ( 'NONE', #9756, #54565, #32663, .T. ) ;
#96752=CIRCLE ( 'NONE', #4809, 0.09999999999999999167 ) ;
#96754=VECTOR ( 'NONE', #86312, 1000.000000000000000 ) ;
#96755=ORIENTED_EDGE ( 'NONE', *, *, #48588, .F. ) ;
#96756=CARTESIAN_POINT ( 'NONE',  ( 0.7999999999999548583, 2.500000000000000000, 4.430127018922196847 ) ) ;
#96757=FACE_OUTER_BOUND ( 'NONE', #93355, .T. ) ;
#96758=CONICAL_SURFACE ( 'NONE', #100983, 0.09999999999999982514, 0.003490658503988666988 ) ;
#96759=VERTEX_POINT ( 'NONE', #66027 ) ;
#96760=DIRECTION ( 'NONE',  ( -0.000000000000000000, -1.000000000000000000, -0.000000000000000000 ) ) ;
#96761=AXIS2_PLACEMENT_3D ( 'NONE', #109818, #60725, #91461 ) ;
#96762=CARTESIAN_POINT ( 'NONE',  ( 4.149999999999939959, 12.50000000000000000, 2.857883832488649301 ) ) ;
#96763=VERTEX_POINT ( 'NONE', #75207 ) ;
#96764=CARTESIAN_POINT ( 'NONE',  ( 4.399999999999940847, 2.500000000000000000, -4.576537180435977348 ) ) ;
#96765=EDGE_LOOP ( 'NONE', ( #104328, #81191, #84265, #70547 ) ) ;
#96766=EDGE_LOOP ( 'NONE', ( #69830, #28558, #126984, #23249 ) ) ;
#96768=ORIENTED_EDGE ( 'NONE', *, *, #103004, .T. ) ;
#96769=FACE_OUTER_BOUND ( 'NONE', #85200, .T. ) ;
#96770=DIRECTION ( 'NONE',  ( -0.000000000000000000, 1.000000000000000000, -0.000000000000000000 ) ) ;
#96771=EDGE_LOOP ( 'NONE', ( #119677, #12354 ) ) ;
#96772=DIRECTION ( 'NONE',  ( -0.000000000000000000, 1.000000000000000000, -0.000000000000000000 ) ) ;
#96773=VERTEX_POINT ( 'NONE', #6428 ) ;
#96774=CARTESIAN_POINT ( 'NONE',  ( 1.449999999999951772, 2.500000000000000000, -6.248780366869526759 ) ) ;
#96775=DIRECTION ( 'NONE',  ( 0.000000000000000000, 0.000000000000000000, 1.000000000000000000 ) ) ;
#96776=FACE_OUTER_BOUND ( 'NONE', #35358, .T. ) ;
#96777=CONICAL_SURFACE ( 'NONE', #15202, 0.1000000000000002554, 0.003490658503988666988 ) ;
#96778=CARTESIAN_POINT ( 'NONE',  ( -8.950000000000008171, 2.500000000000000000, -2.511473670974877948 ) ) ;
#96779=DIRECTION ( 'NONE',  ( -4.274815082592931898E-19, -0.9999939076577903929, -0.003490651415223739937 ) ) ;
#96780=VERTEX_POINT ( 'NONE', #106594 ) ;
#96781=EDGE_CURVE ( 'NONE', #95522, #76489, #3478, .T. ) ;
#96782=VERTEX_POINT ( 'NONE', #86957 ) ;
#96783=CARTESIAN_POINT ( 'NONE',  ( -14.14999999999998614, 12.50000000000000000, -2.922977105672689202 ) ) ;
#96785=CIRCLE ( 'NONE', #86321, 0.1000000000000000472 ) ;
#96786=FACE_OUTER_BOUND ( 'NONE', #3448, .T. ) ;
#96787=VECTOR ( 'NONE', #103768, 1000.000000000000000 ) ;
#96788=DIRECTION ( 'NONE',  ( 0.000000000000000000, 1.000000000000000000, 0.000000000000000000 ) ) ;
#96790=ORIENTED_EDGE ( 'NONE', *, *, #116162, .F. ) ;
#96791=ORIENTED_EDGE ( 'NONE', *, *, #19780, .F. ) ;
#96792=DIRECTION ( 'NONE',  ( 0.000000000000000000, 0.000000000000000000, 1.000000000000000000 ) ) ;
#96793=CARTESIAN_POINT ( 'NONE',  ( 9.349999999999916156, 2.500000000000000000, -2.511473670974877948 ) ) ;
#96794=ADVANCED_FACE ( 'NONE', ( #126894 ), #43208, .T. ) ;
#96795=AXIS2_PLACEMENT_3D ( 'NONE', #87642, #8434, #18902 ) ;
#96796=VECTOR ( 'NONE', #45678, 1000.000000000000000 ) ;
#96797=DIRECTION ( 'NONE',  ( 0.000000000000000000, 0.000000000000000000, 1.000000000000000000 ) ) ;
#96798=CONICAL_SURFACE ( 'NONE', #59273, 0.1000000000000002554, 0.003490658503988666988 ) ;
#96799=SHAPE_DEFINITION_REPRESENTATION ( #12669, #1094 ) ;
#96800=DIRECTION ( 'NONE',  ( 0.000000000000000000, -0.000000000000000000, 1.000000000000000000 ) ) ;
#96802=CARTESIAN_POINT ( 'NONE',  ( -11.84999999999999609, 12.50000000000000000, 2.446380397790835826 ) ) ;
#96803=CIRCLE ( 'NONE', #86337, 0.06509327318403745899 ) ;
#96804=CARTESIAN_POINT ( 'NONE',  ( -3.150000000000029221, 12.50000000000000000, 2.446380397790835826 ) ) ;
#96805=CARTESIAN_POINT ( 'NONE',  ( 11.04999999999990834, 2.500000000000000000, 1.918653347947321564 ) ) ;
#96806=CIRCLE ( 'NONE', #119797, 0.06509327318403745899 ) ;
#96807=EDGE_CURVE ( 'NONE', #40175, #25430, #114202, .T. ) ;
#96808=ADVANCED_FACE ( 'NONE', ( #118998 ), #109160, .T. ) ;
#96809=CARTESIAN_POINT ( 'NONE',  ( 3.349999999999945466, 2.500000000000000000, -6.495190528383302464 ) ) ;
#96810=AXIS2_PLACEMENT_3D ( 'NONE', #7972, #25681, #18445 ) ;
#96811=EDGE_LOOP ( 'NONE', ( #106161, #13619 ) ) ;
#96812=EDGE_CURVE ( 'NONE', #106895, #82230, #105880, .T. ) ;
#96813=CARTESIAN_POINT ( 'NONE',  ( 2.299999999999949640, 2.500000000000000000, -0.2464101615137782308 ) ) ;
#96814=ORIENTED_EDGE ( 'NONE', *, *, #67428, .F. ) ;
#96815=VERTEX_POINT ( 'NONE', #100011 ) ;
#96816=EDGE_CURVE ( 'NONE', #58787, #2492, #122617, .T. ) ;
#96817=DIRECTION ( 'NONE',  ( 0.000000000000000000, 1.000000000000000000, 0.000000000000000000 ) ) ;
#96818=LINE ( 'NONE', #69284, #80375 ) ;
#96819=CARTESIAN_POINT ( 'NONE',  ( 3.349999999999945466, 2.500000000000000000, -2.265063509461101798 ) ) ;
#96820=CIRCLE ( 'NONE', #111494, 0.06509327318403745899 ) ;
#96821=FACE_OUTER_BOUND ( 'NONE', #83210, .T. ) ;
#96822=DIRECTION ( 'NONE',  ( 0.000000000000000000, 0.000000000000000000, 1.000000000000000000 ) ) ;
#96823=FACE_OUTER_BOUND ( 'NONE', #41109, .T. ) ;
#96824=CARTESIAN_POINT ( 'NONE',  ( 12.89999999999989733, 12.50000000000000000, -2.385244779468109755E-15 ) ) ;
#96825=ORIENTED_EDGE ( 'NONE', *, *, #60815, .F. ) ;
#96826=CARTESIAN_POINT ( 'NONE',  ( 14.79999999999989413, 2.500000000000000000, -0.3464101615137782364 ) ) ;
#96827=DIRECTION ( 'NONE',  ( 0.000000000000000000, 0.000000000000000000, -1.000000000000000000 ) ) ;
#96828=VECTOR ( 'NONE', #32396, 1000.000000000000000 ) ;
#96829=EDGE_LOOP ( 'NONE', ( #31521, #81436, #29408, #58043 ) ) ;
#96830=AXIS2_PLACEMENT_3D ( 'NONE', #71783, #1095, #32520 ) ;
#96831=ORIENTED_EDGE ( 'NONE', *, *, #88885, .T. ) ;
#96832=VERTEX_POINT ( 'NONE', #59466 ) ;
#96833=EDGE_LOOP ( 'NONE', ( #108401, #74700 ) ) ;
#96834=EDGE_LOOP ( 'NONE', ( #41919, #8958 ) ) ;
#96835=CONICAL_SURFACE ( 'NONE', #78175, 0.09999999999999999167, 0.003490658503988666988 ) ;
#96836=CARTESIAN_POINT ( 'NONE',  ( 8.299999999999922551, 2.500000000000000000, -4.230127018922201998 ) ) ;
#96837=PLANE ( 'NONE',  #45685 ) ;
#96838=AXIS2_PLACEMENT_3D ( 'NONE', #63987, #6967, #84912 ) ;
#96839=CIRCLE ( 'NONE', #126086, 0.1000000000000000472 ) ;
#96840=ORIENTED_EDGE ( 'NONE', *, *, #30723, .F. ) ;
#96841=CARTESIAN_POINT ( 'NONE',  ( 5.849999999999934808, 2.500000000000000000, -5.902370205355750521 ) ) ;
#96842=CIRCLE ( 'NONE', #119840, 0.09999999999999982514 ) ;
#96843=CARTESIAN_POINT ( 'NONE',  ( -7.900000000000014566, 12.50000000000000000, -4.395220292106239768 ) ) ;
#96845=ORIENTED_EDGE ( 'NONE', *, *, #110020, .F. ) ;
#96846=DIRECTION ( 'NONE',  ( 0.000000000000000000, 0.000000000000000000, -1.000000000000000000 ) ) ;
#96847=EDGE_CURVE ( 'NONE', #13639, #124646, #20209, .T. ) ;
#96848=DIRECTION ( 'NONE',  ( 0.000000000000000000, 1.000000000000000000, 0.000000000000000000 ) ) ;
#96849=ORIENTED_EDGE ( 'NONE', *, *, #118708, .F. ) ;
#96850=CONICAL_SURFACE ( 'NONE', #40450, 0.1000000000000000472, 0.003490658503988666988 ) ;
#96851=AXIS2_PLACEMENT_3D ( 'NONE', #29708, #69628, #50016 ) ;
#96852=AXIS2_PLACEMENT_3D ( 'NONE', #69918, #119014, #37248 ) ;
#96853=ORIENTED_EDGE ( 'NONE', *, *, #33068, .F. ) ;
#96854=EDGE_LOOP ( 'NONE', ( #44928, #86106, #28158, #38776 ) ) ;
#96855=CARTESIAN_POINT ( 'NONE',  ( 8.949999999999921130, 2.500000000000000000, -6.841600689897078702 ) ) ;
#96856=EDGE_CURVE ( 'NONE', #96782, #100782, #116330, .T. ) ;
#96857=AXIS2_PLACEMENT_3D ( 'NONE', #27210, #35752, #75657 ) ;
#96858=EDGE_CURVE ( 'NONE', #9937, #79720, #110003, .T. ) ;
#96859=ADVANCED_FACE ( 'NONE', ( #97418 ), #40461, .T. ) ;
#96860=DIRECTION ( 'NONE',  ( 0.000000000000000000, 1.000000000000000000, 0.000000000000000000 ) ) ;
#96861=EDGE_CURVE ( 'NONE', #95073, #16529, #32745, .T. ) ;
#96862=VERTEX_POINT ( 'NONE', #118349 ) ;
#96863=CARTESIAN_POINT ( 'NONE',  ( -3.950000000000028155, 2.500000000000000000, -6.841600689897077814 ) ) ;
#96864=DIRECTION ( 'NONE',  ( -4.274815082592931898E-19, -0.9999939076577903929, -0.003490651415223739937 ) ) ;
#96865=DIRECTION ( 'NONE',  ( 0.000000000000000000, 0.000000000000000000, -1.000000000000000000 ) ) ;
#96866=DIRECTION ( 'NONE',  ( -0.000000000000000000, -1.000000000000000000, -0.000000000000000000 ) ) ;
#96867=EDGE_CURVE ( 'NONE', #98786, #46014, #49471, .T. ) ;
#96868=ORIENTED_EDGE ( 'NONE', *, *, #126017, .T. ) ;
#96869=ADVANCED_FACE ( 'NONE', ( #29990 ), #87004, .T. ) ;
#96870=DIRECTION ( 'NONE',  ( 0.000000000000000000, 0.000000000000000000, -1.000000000000000000 ) ) ;
#96871=EDGE_LOOP ( 'NONE', ( #86167, #48507 ) ) ;
#96872=EDGE_LOOP ( 'NONE', ( #24637, #128405, #121358, #51453 ) ) ;
#96873=CONICAL_SURFACE ( 'NONE', #113610, 0.09999999999999982514, 0.003490658503988666988 ) ;
#96874=VERTEX_POINT ( 'NONE', #79090 ) ;
#96875=AXIS2_PLACEMENT_3D ( 'NONE', #656, #52993, #101447 ) ;
#96876=FACE_OUTER_BOUND ( 'NONE', #104093, .T. ) ;
#96877=FACE_BOUND ( 'NONE', #100809, .T. ) ;
#96878=DIRECTION ( 'NONE',  ( 0.000000000000000000, 0.000000000000000000, 1.000000000000000000 ) ) ;
#96879=LINE ( 'NONE', #117798, #96655 ) ;
#96880=DIRECTION ( 'NONE',  ( -0.000000000000000000, 1.000000000000000000, -0.000000000000000000 ) ) ;
#96882=AXIS2_PLACEMENT_3D ( 'NONE', #98274, #87804, #127745 ) ;
#96883=CONICAL_SURFACE ( 'NONE', #52983, 0.1000000000000002554, 0.003490658503988666988 ) ;
#96884=AXIS2_PLACEMENT_3D ( 'NONE', #45624, #94700, #36454 ) ;
#96885=AXIS2_PLACEMENT_3D ( 'NONE', #20544, #120677, #31649 ) ;
#96886=ORIENTED_EDGE ( 'NONE', *, *, #11487, .T. ) ;
#96887=DIRECTION ( 'NONE',  ( 0.000000000000000000, 1.000000000000000000, 0.000000000000000000 ) ) ;
#96888=DIRECTION ( 'NONE',  ( 0.000000000000000000, 0.000000000000000000, -1.000000000000000000 ) ) ;
#96889=EDGE_CURVE ( 'NONE', #47981, #64551, #7746, .T. ) ;
#96890=CARTESIAN_POINT ( 'NONE',  ( -8.750000000000010658, 12.50000000000000000, 2.922977105672686982 ) ) ;
#96891=LINE ( 'NONE', #45230, #82378 ) ;
#96892=ORIENTED_EDGE ( 'NONE', *, *, #82414, .T. ) ;
#96893=AXIS2_PLACEMENT_3D ( 'NONE', #50493, #41976, #2667 ) ;
#96894=CARTESIAN_POINT ( 'NONE',  ( -0.8500000000000386136, 12.50000000000000000, 2.792790559304612064 ) ) ;
#96895=CIRCLE ( 'NONE', #25803, 0.06509327318403745899 ) ;
#96896=CIRCLE ( 'NONE', #44685, 0.06509327318403745899 ) ;
#96897=CARTESIAN_POINT ( 'NONE',  ( -5.850000000000019185, 2.500000000000000000, 2.165063509461097713 ) ) ;
#96898=EDGE_LOOP ( 'NONE', ( #117473, #61644 ) ) ;
#96899=VECTOR ( 'NONE', #75258, 1000.000000000000000 ) ;
#96900=DIRECTION ( 'NONE',  ( -0.000000000000000000, 1.000000000000000000, -0.000000000000000000 ) ) ;
#96901=DIRECTION ( 'NONE',  ( -0.000000000000000000, 1.000000000000000000, -0.000000000000000000 ) ) ;
#96902=FACE_BOUND ( 'NONE', #5283, .T. ) ;
#96903=CARTESIAN_POINT ( 'NONE',  ( -6.050000000000022027, 2.500000000000000000, -1.918653347947326004 ) ) ;
#96904=ORIENTED_EDGE ( 'NONE', *, *, #25524, .F. ) ;
#96905=DIRECTION ( 'NONE',  ( 0.000000000000000000, -0.9999939076577903929, 0.003490651415223739937 ) ) ;
#96906=ORIENTED_EDGE ( 'NONE', *, *, #116910, .T. ) ;
#96907=ORIENTED_EDGE ( 'NONE', *, *, #11734, .T. ) ;
#96908=CARTESIAN_POINT ( 'NONE',  ( 17.91370874550468884, 0.4812889678260186543, -4.985910759330088204 ) ) ;
#96910=VECTOR ( 'NONE', #93676, 1000.000000000000000 ) ;
#96911=ORIENTED_EDGE ( 'NONE', *, *, #89063, .T. ) ;
#96913=FACE_OUTER_BOUND ( 'NONE', #56625, .T. ) ;
#96914=EDGE_CURVE ( 'NONE', #76856, #34681, #15978, .T. ) ;
#96915=DIRECTION ( 'NONE',  ( 0.000000000000000000, -0.000000000000000000, 1.000000000000000000 ) ) ;
#96916=DIRECTION ( 'NONE',  ( 0.000000000000000000, 1.000000000000000000, 0.000000000000000000 ) ) ;
#96917=CIRCLE ( 'NONE', #67673, 0.1000000000000002554 ) ;
#96918=CONICAL_SURFACE ( 'NONE', #71910, 0.09999999999999999167, 0.003490658503988666988 ) ;
#96919=VECTOR ( 'NONE', #25233, 1000.000000000000000 ) ;
#96920=ORIENTED_EDGE ( 'NONE', *, *, #53892, .F. ) ;
#96921=FACE_OUTER_BOUND ( 'NONE', #100847, .T. ) ;
#96922=LINE ( 'NONE', #87103, #106142 ) ;
#96923=FACE_OUTER_BOUND ( 'NONE', #86746, .T. ) ;
#96924=CARTESIAN_POINT ( 'NONE',  ( -8.350000000000013856, 2.500000000000000000, -5.702370205355745014 ) ) ;
#96925=ORIENTED_EDGE ( 'NONE', *, *, #58871, .F. ) ;
#96926=CARTESIAN_POINT ( 'NONE',  ( -10.00000000000000355, 2.500000000000000000, 3.637306695894644726 ) ) ;
#96927=VERTEX_POINT ( 'NONE', #108535 ) ;
#96928=VECTOR ( 'NONE', #52158, 1000.000000000000000 ) ;
#96929=CARTESIAN_POINT ( 'NONE',  ( 1.249999999999953815, 12.50000000000000000, -2.857883832488653741 ) ) ;
#96930=DIRECTION ( 'NONE',  ( 0.000000000000000000, 0.000000000000000000, 1.000000000000000000 ) ) ;
#96931=VECTOR ( 'NONE', #122119, 1000.000000000000000 ) ;
#96932=ORIENTED_EDGE ( 'NONE', *, *, #125927, .F. ) ;
#96933=VECTOR ( 'NONE', #123998, 1000.000000000000000 ) ;
#96934=CARTESIAN_POINT ( 'NONE',  ( 13.94999999999989626, 2.500000000000000000, 2.511473670974873507 ) ) ;
#96935=PLANE ( 'NONE',  #39043 ) ;
#96936=FACE_OUTER_BOUND ( 'NONE', #112281, .T. ) ;
#96937=DIRECTION ( 'NONE',  ( 0.000000000000000000, 1.000000000000000000, 0.000000000000000000 ) ) ;
#96938=EDGE_LOOP ( 'NONE', ( #6292, #24130 ) ) ;
#96939=CARTESIAN_POINT ( 'NONE',  ( -2.900000000000030109, 2.500000000000000000, 0.6928203230275494784 ) ) ;
#96940=DIRECTION ( 'NONE',  ( 0.000000000000000000, -0.9999939076577903929, 0.003490651415223739937 ) ) ;
#96941=DIRECTION ( 'NONE',  ( 0.000000000000000000, 1.000000000000000000, 0.000000000000000000 ) ) ;
#96942=CARTESIAN_POINT ( 'NONE',  ( 8.749999999999920064, 12.50000000000000000, 5.802370205355744659 ) ) ;
#96943=AXIS2_PLACEMENT_3D ( 'NONE', #118197, #79568, #128698 ) ;
#96945=ORIENTED_EDGE ( 'NONE', *, *, #113217, .F. ) ;
#96946=VERTEX_POINT ( 'NONE', #128186 ) ;
#96948=CIRCLE ( 'NONE', #122100, 0.1000000000000002554 ) ;
#96949=ORIENTED_EDGE ( 'NONE', *, *, #108531, .T. ) ;
#96950=AXIS2_PLACEMENT_3D ( 'NONE', #61101, #41489, #121309 ) ;
#96951=CIRCLE ( 'NONE', #23806, 0.1000000000000000472 ) ;
#96952=CARTESIAN_POINT ( 'NONE',  ( 7.699999999999925571, 2.500000000000000000, -4.776537180435978414 ) ) ;
#96953=VERTEX_POINT ( 'NONE', #70539 ) ;
#96954=ORIENTED_EDGE ( 'NONE', *, *, #81640, .T. ) ;
#96955=EDGE_LOOP ( 'NONE', ( #6540, #124870 ) ) ;
#96956=AXIS2_PLACEMENT_3D ( 'NONE', #57817, #117337, #109492 ) ;
#96957=CARTESIAN_POINT ( 'NONE',  ( -8.150000000000012790, 2.500000000000000000, 1.818653347947321475 ) ) ;
#96958=CIRCLE ( 'NONE', #9137, 0.06509327318403745899 ) ;
#96959=CARTESIAN_POINT ( 'NONE',  ( 13.94999999999989271, 2.500000000000000000, -1.918653347947326004 ) ) ;
#96960=EDGE_CURVE ( 'NONE', #69282, #21419, #97474, .T. ) ;
#96961=DIRECTION ( 'NONE',  ( 0.000000000000000000, -0.9999939076577903929, 0.003490651415223739937 ) ) ;
#96962=CARTESIAN_POINT ( 'NONE',  ( -12.89999999999999325, 2.500000000000000000, 0.6928203230275535862 ) ) ;
#96963=FACE_OUTER_BOUND ( 'NONE', #102551, .T. ) ;
#96964=FACE_OUTER_BOUND ( 'NONE', #5876, .T. ) ;
#96965=ADVANCED_FACE ( 'NONE', ( #109828 ), #30596, .T. ) ;
#96966=ORIENTED_EDGE ( 'NONE', *, *, #47914, .T. ) ;
#96967=ADVANCED_FACE ( 'NONE', ( #60103 ), #18856, .T. ) ;
#96968=CARTESIAN_POINT ( 'NONE',  ( 4.599999999999939249, 2.500000000000000000, -3.637306695894650055 ) ) ;
#96969=ORIENTED_EDGE ( 'NONE', *, *, #11695, .T. ) ;
#96970=ORIENTED_EDGE ( 'NONE', *, *, #76594, .F. ) ;
#96971=ORIENTED_EDGE ( 'NONE', *, *, #5373, .F. ) ;
#96972=EDGE_LOOP ( 'NONE', ( #43950, #73377 ) ) ;
#96974=CARTESIAN_POINT ( 'NONE',  ( -10.85000000000000142, 2.500000000000000000, -5.802370205355746435 ) ) ;
#96975=EDGE_CURVE ( 'NONE', #56893, #121027, #1320, .T. ) ;
#96976=AXIS2_PLACEMENT_3D ( 'NONE', #42425, #14219, #54171 ) ;
#96977=CONICAL_SURFACE ( 'NONE', #115749, 0.1000000000000000056, 0.003490658503988666988 ) ;
#96978=EDGE_CURVE ( 'NONE', #119499, #123701, #82907, .T. ) ;
#96979=ORIENTED_EDGE ( 'NONE', *, *, #69841, .T. ) ;
#96980=ORIENTED_EDGE ( 'NONE', *, *, #48218, .F. ) ;
#96981=EDGE_CURVE ( 'NONE', #95501, #80857, #55698, .T. ) ;
#96982=AXIS2_PLACEMENT_3D ( 'NONE', #71604, #70964, #111534 ) ;
#96983=CARTESIAN_POINT ( 'NONE',  ( 4.599999999999938360, 2.500000000000000000, -2.276824562219559311E-15 ) ) ;
#96984=VECTOR ( 'NONE', #82861, 1000.000000000000000 ) ;
#96985=DIRECTION ( 'NONE',  ( 0.000000000000000000, 1.000000000000000000, 0.000000000000000000 ) ) ;
#96986=AXIS2_PLACEMENT_3D ( 'NONE', #107658, #57917, #50663 ) ;
#96987=CARTESIAN_POINT ( 'NONE',  ( -11.89999999999999680, 2.500000000000000000, -4.083716857408424161 ) ) ;
#96989=AXIS2_PLACEMENT_3D ( 'NONE', #60606, #42243, #80881 ) ;
#96990=AXIS2_PLACEMENT_3D ( 'NONE', #127130, #119225, #118570 ) ;
#96991=DIRECTION ( 'NONE',  ( 0.000000000000000000, -0.000000000000000000, 1.000000000000000000 ) ) ;
#96992=ORIENTED_EDGE ( 'NONE', *, *, #35268, .T. ) ;
#96993=ADVANCED_FACE ( 'NONE', ( #31282 ), #9741, .T. ) ;
#96994=CARTESIAN_POINT ( 'NONE',  ( 8.149999999999920419, 2.500000000000000000, 6.248780366869521430 ) ) ;
#96995=ORIENTED_EDGE ( 'NONE', *, *, #28106, .F. ) ;
#96996=PLANE ( 'NONE',  #84028 ) ;
#96997=CIRCLE ( 'NONE', #86528, 0.1000000000000002554 ) ;
#96998=ORIENTED_EDGE ( 'NONE', *, *, #70120, .T. ) ;
#96999=DIRECTION ( 'NONE',  ( 0.000000000000000000, 0.000000000000000000, -1.000000000000000000 ) ) ;
#97000=ORIENTED_EDGE ( 'NONE', *, *, #92127, .T. ) ;
#97001=AXIS2_PLACEMENT_3D ( 'NONE', #41167, #21499, #61444 ) ;
#97002=ORIENTED_EDGE ( 'NONE', *, *, #19223, .T. ) ;
#97004=PLANE ( 'NONE',  #4594 ) ;
#97005=LINE ( 'NONE', #83501, #113544 ) ;
#97006=DIRECTION ( 'NONE',  ( -0.000000000000000000, -1.000000000000000000, -0.000000000000000000 ) ) ;
#97007=PLANE ( 'NONE',  #120273 ) ;
#97008=ORIENTED_EDGE ( 'NONE', *, *, #57355, .F. ) ;
#97009=LINE ( 'NONE', #19071, #62431 ) ;
#97010=CARTESIAN_POINT ( 'NONE',  ( -4.550000000000022915, 12.50000000000000000, -2.165063509461101710 ) ) ;
#97011=ADVANCED_FACE ( 'NONE', ( #3104 ), #64026, .T. ) ;
#97012=DIRECTION ( 'NONE',  ( 0.000000000000000000, 0.000000000000000000, 1.000000000000000000 ) ) ;
#97013=DIRECTION ( 'NONE',  ( 0.000000000000000000, 0.000000000000000000, 1.000000000000000000 ) ) ;
#97014=AXIS2_PLACEMENT_3D ( 'NONE', #35825, #78342, #58053 ) ;
#97015=CARTESIAN_POINT ( 'NONE',  ( -7.300000000000016698, 2.500000000000000000, -4.676537180435978769 ) ) ;
#97016=ORIENTED_EDGE ( 'NONE', *, *, #44435, .F. ) ;
#97017=VERTEX_POINT ( 'NONE', #113040 ) ;
#97018=ADVANCED_FACE ( 'NONE', ( #31916 ), #21438, .T. ) ;
#97019=PLANE ( 'NONE',  #54799 ) ;
#97020=ADVANCED_FACE ( 'NONE', ( #73750 ), #80764, .T. ) ;
#97021=EDGE_CURVE ( 'NONE', #105515, #42013, #82953, .T. ) ;
#97022=ORIENTED_EDGE ( 'NONE', *, *, #91887, .T. ) ;
#97023=CONICAL_SURFACE ( 'NONE', #69837, 0.1000000000000002554, 0.003490658503988666988 ) ;
#97024=CARTESIAN_POINT ( 'NONE',  ( 4.349999999999936584, 12.50000000000000000, 6.213873640053558134 ) ) ;
#97025=DIRECTION ( 'NONE',  ( 0.000000000000000000, -0.9999939076577903929, 0.003490651415223739937 ) ) ;
#97026=EDGE_CURVE ( 'NONE', #9406, #26024, #7575, .T. ) ;
#97027=EDGE_CURVE ( 'NONE', #19044, #111256, #18039, .T. ) ;
#97028=ORIENTED_EDGE ( 'NONE', *, *, #73953, .F. ) ;
#97030=DIRECTION ( 'NONE',  ( 0.000000000000000000, 1.000000000000000000, 0.000000000000000000 ) ) ;
#97031=DIRECTION ( 'NONE',  ( 0.000000000000000000, 0.000000000000000000, 1.000000000000000000 ) ) ;
#97032=EDGE_CURVE ( 'NONE', #37015, #114052, #51514, .T. ) ;
#97033=PLANE ( 'NONE',  #64947 ) ;
#97034=DIRECTION ( 'NONE',  ( 0.000000000000000000, -0.9999939076577903929, 0.003490651415223739937 ) ) ;
#97036=EDGE_CURVE ( 'NONE', #126646, #65379, #124672, .T. ) ;
#97037=ADVANCED_FACE ( 'NONE', ( #93409 ), #13932, .T. ) ;
#97038=CIRCLE ( 'NONE', #115898, 0.06509327318403745899 ) ;
#97039=EDGE_CURVE ( 'NONE', #100363, #124, #28524, .T. ) ;
#97040=CARTESIAN_POINT ( 'NONE',  ( -10.65000000000000391, 2.500000000000000000, -6.741600689897074616 ) ) ;
#97041=CARTESIAN_POINT ( 'NONE',  ( 11.24999999999990941, 12.50000000000000000, 7.188010851410848723 ) ) ;
#97042=ORIENTED_EDGE ( 'NONE', *, *, #39582, .T. ) ;
#97043=CARTESIAN_POINT ( 'NONE',  ( 3.749999999999942268, 12.50000000000000000, -5.867463478539787225 ) ) ;
#97044=DIRECTION ( 'NONE',  ( 0.000000000000000000, 0.000000000000000000, 1.000000000000000000 ) ) ;
#97045=EDGE_CURVE ( 'NONE', #54254, #95676, #120549, .T. ) ;
#97046=CARTESIAN_POINT ( 'NONE',  ( -15.79999999999998117, 12.50000000000000000, 0.000000000000000000 ) ) ;
#97047=ORIENTED_EDGE ( 'NONE', *, *, #31422, .T. ) ;
#97048=AXIS2_PLACEMENT_3D ( 'NONE', #5284, #105441, #103506 ) ;
#97049=AXIS2_PLACEMENT_3D ( 'NONE', #32211, #121850, #102224 ) ;
#97051=CIRCLE ( 'NONE', #40651, 0.06509327318403745899 ) ;
#97052=VERTEX_POINT ( 'NONE', #102569 ) ;
#97053=DIRECTION ( 'NONE',  ( 0.000000000000000000, -0.000000000000000000, 1.000000000000000000 ) ) ;
#97054=CARTESIAN_POINT ( 'NONE',  ( 16.55874544816229132, -0.4845305829427751232, 6.091953208798936537 ) ) ;
#97055=DIRECTION ( 'NONE',  ( -0.000000000000000000, -1.000000000000000000, -0.000000000000000000 ) ) ;
#97056=CONICAL_SURFACE ( 'NONE', #7157, 0.09999999999999982514, 0.003490658503988666988 ) ;
#97057=ORIENTED_EDGE ( 'NONE', *, *, #77601, .T. ) ;
#97058=CARTESIAN_POINT ( 'NONE',  ( -8.350000000000012079, 2.500000000000000000, -2.857883832488653741 ) ) ;
#97059=DIRECTION ( 'NONE',  ( 0.000000000000000000, 0.000000000000000000, 1.000000000000000000 ) ) ;
#97060=ORIENTED_EDGE ( 'NONE', *, *, #81738, .T. ) ;
#97061=DIRECTION ( 'NONE',  ( 0.000000000000000000, 0.000000000000000000, 1.000000000000000000 ) ) ;
#97062=EDGE_LOOP ( 'NONE', ( #30156, #115109 ) ) ;
#97064=VERTEX_POINT ( 'NONE', #92106 ) ;
#97065=CARTESIAN_POINT ( 'NONE',  ( 11.84999999999990727, 2.500000000000000000, -2.411473670974877859 ) ) ;
#97066=CARTESIAN_POINT ( 'NONE',  ( 5.199999999999933564, 2.500000000000000000, 4.083716857408420609 ) ) ;
#97067=AXIS2_PLACEMENT_3D ( 'NONE', #8910, #109717, #120176 ) ;
#97068=AXIS2_PLACEMENT_3D ( 'NONE', #77139, #96760, #88896 ) ;
#97069=VERTEX_POINT ( 'NONE', #12886 ) ;
#97070=EDGE_LOOP ( 'NONE', ( #8936, #57996 ) ) ;
#97071=DIRECTION ( 'NONE',  ( 0.000000000000000000, 1.000000000000000000, 0.000000000000000000 ) ) ;
#97072=DIRECTION ( 'NONE',  ( -0.000000000000000000, 1.000000000000000000, -0.000000000000000000 ) ) ;
#97073=VERTEX_POINT ( 'NONE', #42382 ) ;
#97074=DIRECTION ( 'NONE',  ( -0.000000000000000000, -1.000000000000000000, -0.000000000000000000 ) ) ;
#97075=CIRCLE ( 'NONE', #933, 0.09999999999999982514 ) ;
#97077=CIRCLE ( 'NONE', #32361, 0.06509327318403745899 ) ;
#97078=EDGE_CURVE ( 'NONE', #39808, #106452, #80852, .T. ) ;
#97079=CIRCLE ( 'NONE', #128498, 0.09999999999999982514 ) ;
#97080=LINE ( 'NONE', #7391, #20041 ) ;
#97081=CARTESIAN_POINT ( 'NONE',  ( 11.44999999999991047, 2.500000000000000000, 6.248780366869520542 ) ) ;
#97082=CARTESIAN_POINT ( 'NONE',  ( 11.64999999999990266, 2.500000000000000000, 2.265063509461097357 ) ) ;
#97083=CARTESIAN_POINT ( 'NONE',  ( -9.400000000000009237, 12.50000000000000000, -3.983716857408421852 ) ) ;
#97084=CIRCLE ( 'NONE', #111673, 0.09999999999999999167 ) ;
#97085=CIRCLE ( 'NONE', #63653, 0.1000000000000000472 ) ;
#97086=ORIENTED_EDGE ( 'NONE', *, *, #7640, .F. ) ;
#97087=VERTEX_POINT ( 'NONE', #72492 ) ;
#97088=VERTEX_POINT ( 'NONE', #123499 ) ;
#97089=ORIENTED_EDGE ( 'NONE', *, *, #4058, .F. ) ;
#97090=DIRECTION ( 'NONE',  ( -0.000000000000000000, -1.000000000000000000, -0.000000000000000000 ) ) ;
#97091=CARTESIAN_POINT ( 'NONE',  ( -11.84999999999999609, 12.50000000000000000, 2.511473670974873507 ) ) ;
#97092=AXIS2_PLACEMENT_3D ( 'NONE', #88116, #65274, #115666 ) ;
#97093=CARTESIAN_POINT ( 'NONE',  ( -14.59999999999998366, 12.50000000000000000, 0.06509327318403732021 ) ) ;
#97094=VERTEX_POINT ( 'NONE', #33837 ) ;
#97095=EDGE_CURVE ( 'NONE', #50837, #77356, #68313, .T. ) ;
#97096=FACE_BOUND ( 'NONE', #114559, .T. ) ;
#97097=DIRECTION ( 'NONE',  ( 0.000000000000000000, -0.9999939076577903929, 0.003490651415223739937 ) ) ;
#97098=DIRECTION ( 'NONE',  ( 0.000000000000000000, 1.000000000000000000, 0.000000000000000000 ) ) ;
#97099=CARTESIAN_POINT ( 'NONE',  ( 1.449999999999952216, 12.50000000000000000, 1.818653347947321475 ) ) ;
#97100=CARTESIAN_POINT ( 'NONE',  ( -2.050000000000033129, 12.50000000000000000, 6.430097255199259010 ) ) ;
#97101=CARTESIAN_POINT ( 'NONE',  ( 14.54999999999989591, 2.500000000000000000, 2.165063509461097713 ) ) ;
#97102=DIRECTION ( 'NONE',  ( -0.000000000000000000, 1.000000000000000000, -0.000000000000000000 ) ) ;
#97103=DIRECTION ( 'NONE',  ( 0.000000000000000000, -0.000000000000000000, 1.000000000000000000 ) ) ;
#97104=DIRECTION ( 'NONE',  ( 0.000000000000000000, 0.000000000000000000, -1.000000000000000000 ) ) ;
#97105=DIRECTION ( 'NONE',  ( 0.000000000000000000, -0.9999939076577903929, 0.003490651415223739937 ) ) ;
#97106=AXIS2_PLACEMENT_3D ( 'NONE', #37539, #117335, #106897 ) ;
#97107=DIRECTION ( 'NONE',  ( 0.000000000000000000, -0.000000000000000000, 1.000000000000000000 ) ) ;
#97108=EDGE_LOOP ( 'NONE', ( #51349, #39528 ) ) ;
#97109=ORIENTED_EDGE ( 'NONE', *, *, #76209, .T. ) ;
#97110=EDGE_LOOP ( 'NONE', ( #128290, #19482 ) ) ;
#97111=VERTEX_POINT ( 'NONE', #16752 ) ;
#97112=CARTESIAN_POINT ( 'NONE',  ( 10.19999999999991047, 12.50000000000000000, -3.983716857408426293 ) ) ;
#97113=CARTESIAN_POINT ( 'NONE',  ( -14.19999999999998685, 2.500000000000000000, -1.084202172485504434E-16 ) ) ;
#97114=EDGE_LOOP ( 'NONE', ( #78899, #93127 ) ) ;
#97115=ORIENTED_EDGE ( 'NONE', *, *, #50620, .T. ) ;
#97116=ORIENTED_EDGE ( 'NONE', *, *, #117678, .T. ) ;
#97117=DIRECTION ( 'NONE',  ( 0.000000000000000000, 1.000000000000000000, 0.000000000000000000 ) ) ;
#97118=AXIS2_PLACEMENT_3D ( 'NONE', #85502, #4991, #37062 ) ;
#97119=VECTOR ( 'NONE', #13002, 1000.000000000000000 ) ;
#97120=EDGE_CURVE ( 'NONE', #99960, #38921, #64109, .T. ) ;
#97121=CARTESIAN_POINT ( 'NONE',  ( 4.849235612605155232, -2.500000000000000888, 8.943930330503281567 ) ) ;
#97122=CARTESIAN_POINT ( 'NONE',  ( -3.750000000000029310, 12.50000000000000000, -7.122917578226816815 ) ) ;
#97123=LINE ( 'NONE', #47389, #103634 ) ;
#97124=LINE ( 'NONE', #25809, #102053 ) ;
#97125=EDGE_LOOP ( 'NONE', ( #84617, #53475 ) ) ;
#97126=EDGE_CURVE ( 'NONE', #102170, #77027, #57868, .T. ) ;
#97127=CARTESIAN_POINT ( 'NONE',  ( 8.099999999999923261, 12.50000000000000000, 4.676537180435972552 ) ) ;
#97128=ORIENTED_EDGE ( 'NONE', *, *, #87672, .T. ) ;
#97129=AXIS2_PLACEMENT_3D ( 'NONE', #8010, #7359, #46026 ) ;
#97130=ORIENTED_EDGE ( 'NONE', *, *, #19611, .T. ) ;
#97131=VERTEX_POINT ( 'NONE', #56678 ) ;
#97132=VECTOR ( 'NONE', #28189, 1000.000000000000000 ) ;
#97133=ADVANCED_FACE ( 'NONE', ( #64583 ), #105972, .T. ) ;
#97134=CARTESIAN_POINT ( 'NONE',  ( 2.899999999999944844, 2.500000000000000000, 5.122947341949749323 ) ) ;
#97135=EDGE_CURVE ( 'NONE', #89102, #77185, #32829, .T. ) ;
#97136=EDGE_CURVE ( 'NONE', #70290, #15958, #46894, .T. ) ;
#97137=ORIENTED_EDGE ( 'NONE', *, *, #10675, .F. ) ;
#97138=ADVANCED_FACE ( 'NONE', ( #85518 ), #37024, .T. ) ;
#97139=EDGE_CURVE ( 'NONE', #37274, #79643, #85032, .T. ) ;
#97140=ORIENTED_EDGE ( 'NONE', *, *, #58152, .F. ) ;
#97141=CARTESIAN_POINT ( 'NONE',  ( -5.000000000000023093, 2.500000000000000000, 5.022947341949748790 ) ) ;
#97142=DIRECTION ( 'NONE',  ( 0.000000000000000000, 0.000000000000000000, -1.000000000000000000 ) ) ;
#97143=CARTESIAN_POINT ( 'NONE',  ( -3.550000000000030909, 2.500000000000000000, -6.841600689897078702 ) ) ;
#97144=DIRECTION ( 'NONE',  ( 0.000000000000000000, 0.000000000000000000, 1.000000000000000000 ) ) ;
#97145=DIRECTION ( 'NONE',  ( 0.000000000000000000, 1.000000000000000000, 0.000000000000000000 ) ) ;
#97146=AXIS2_PLACEMENT_3D ( 'NONE', #107071, #57344, #64577 ) ;
#97147=EDGE_CURVE ( 'NONE', #113918, #63903, #44963, .T. ) ;
#97148=ORIENTED_EDGE ( 'NONE', *, *, #120225, .T. ) ;
#97149=AXIS2_PLACEMENT_3D ( 'NONE', #97226, #8192, #118152 ) ;
#97150=LINE ( 'NONE', #118071, #21978 ) ;
#97151=EDGE_CURVE ( 'NONE', #37202, #64313, #49553, .T. ) ;
#97152=EDGE_CURVE ( 'NONE', #53990, #5536, #56045, .T. ) ;
#97153=EDGE_LOOP ( 'NONE', ( #71119, #11302 ) ) ;
#97154=LINE ( 'NONE', #127269, #94310 ) ;
#97155=ORIENTED_EDGE ( 'NONE', *, *, #95780, .F. ) ;
#97156=DIRECTION ( 'NONE',  ( 0.000000000000000000, 1.000000000000000000, 0.000000000000000000 ) ) ;
#97157=CARTESIAN_POINT ( 'NONE',  ( 21.25101288990114767, 0.2446430927199364502, -4.189229928197901742 ) ) ;
#97158=ORIENTED_EDGE ( 'NONE', *, *, #13615, .T. ) ;
#97159=DIRECTION ( 'NONE',  ( 0.000000000000000000, 0.000000000000000000, -1.000000000000000000 ) ) ;
#97160=DIRECTION ( 'NONE',  ( 0.000000000000000000, 1.000000000000000000, 0.000000000000000000 ) ) ;
#97161=ORIENTED_EDGE ( 'NONE', *, *, #60269, .T. ) ;
#97162=CIRCLE ( 'NONE', #17721, 0.1000000000000002554 ) ;
#97163=DIRECTION ( 'NONE',  ( -0.000000000000000000, 1.000000000000000000, -0.000000000000000000 ) ) ;
#97164=ORIENTED_EDGE ( 'NONE', *, *, #54550, .T. ) ;
#97165=CIRCLE ( 'NONE', #32357, 0.1000000000000002554 ) ;
#97166=VERTEX_POINT ( 'NONE', #35153 ) ;
#97167=CARTESIAN_POINT ( 'NONE',  ( 5.449999999999936229, 12.50000000000000000, -2.165063509461101710 ) ) ;
#97168=LINE ( 'NONE', #7488, #1215 ) ;
#97170=DIRECTION ( 'NONE',  ( 0.000000000000000000, -0.000000000000000000, 1.000000000000000000 ) ) ;
#97171=AXIS2_PLACEMENT_3D ( 'NONE', #57383, #55448, #126117 ) ;
#97172=DIRECTION ( 'NONE',  ( 0.000000000000000000, 0.000000000000000000, 1.000000000000000000 ) ) ;
#97173=VECTOR ( 'NONE', #11121, 1000.000000000000000 ) ;
#97174=AXIS2_PLACEMENT_3D ( 'NONE', #28416, #68326, #58531 ) ;
#97175=CARTESIAN_POINT ( 'NONE',  ( -6.700000000000016165, 2.500000000000000000, 4.330127018922196314 ) ) ;
#97176=AXIS2_PLACEMENT_3D ( 'NONE', #20724, #88811, #41674 ) ;
#97177=VERTEX_POINT ( 'NONE', #14813 ) ;
#97178=AXIS2_PLACEMENT_3D ( 'NONE', #64633, #95389, #114372 ) ;
#97179=CARTESIAN_POINT ( 'NONE',  ( 32.27759793366435304, 1.406472199115788468, -4.686460523057745853 ) ) ;
#97180=CARTESIAN_POINT ( 'NONE',  ( 1.649999999999949729, 12.50000000000000000, 7.188010851410848723 ) ) ;
#97182=VERTEX_POINT ( 'NONE', #24032 ) ;
#97183=CONICAL_SURFACE ( 'NONE', #97092, 0.1000000000000002554, 0.003490658503988666988 ) ;
#97184=DIRECTION ( 'NONE',  ( 0.000000000000000000, 0.000000000000000000, 1.000000000000000000 ) ) ;
#97185=CARTESIAN_POINT ( 'NONE',  ( 8.549999999999920774, 2.500000000000000000, -2.511473670974877948 ) ) ;
#97186=CARTESIAN_POINT ( 'NONE',  ( -12.89999999999999147, 12.50000000000000000, 4.957854068765711553 ) ) ;
#97187=EDGE_CURVE ( 'NONE', #26124, #80887, #103831, .T. ) ;
#97188=CARTESIAN_POINT ( 'NONE',  ( 3.949999999999939782, 12.50000000000000000, 2.446380397790835826 ) ) ;
#97189=CARTESIAN_POINT ( 'NONE',  ( -5.000000000000024869, 12.50000000000000000, -5.022947341949754119 ) ) ;
#97190=EDGE_LOOP ( 'NONE', ( #76500, #95843, #53496, #71616 ) ) ;
#97191=EDGE_CURVE ( 'NONE', #109936, #81547, #62076, .T. ) ;
#97192=ADVANCED_FACE ( 'NONE', ( #84217 ), #55802, .T. ) ;
#97193=CARTESIAN_POINT ( 'NONE',  ( -11.84999999999999787, 2.500000000000000000, -2.411473670974874306 ) ) ;
#97194=CARTESIAN_POINT ( 'NONE',  ( 0.8499999999999553468, 2.500000000000000000, -2.165063509461101710 ) ) ;
#97195=AXIS2_PLACEMENT_3D ( 'NONE', #66334, #68912, #9999 ) ;
#97197=EDGE_CURVE ( 'NONE', #73967, #49583, #16107, .T. ) ;
#97198=LINE ( 'NONE', #8162, #46874 ) ;
#97199=ORIENTED_EDGE ( 'NONE', *, *, #83616, .T. ) ;
#97201=ORIENTED_EDGE ( 'NONE', *, *, #37782, .F. ) ;
#97202=FACE_OUTER_BOUND ( 'NONE', #114178, .T. ) ;
#97203=ORIENTED_EDGE ( 'NONE', *, *, #117314, .T. ) ;
#97204=EDGE_CURVE ( 'NONE', #115693, #111656, #26557, .T. ) ;
#97205=DIRECTION ( 'NONE',  ( 0.000000000000000000, 1.000000000000000000, 0.000000000000000000 ) ) ;
#97206=DIRECTION ( 'NONE',  ( -4.274815082592931898E-19, -0.9999939076577903929, -0.003490651415223739937 ) ) ;
#97207=DIRECTION ( 'NONE',  ( -4.274815082592931898E-19, -0.9999939076577903929, -0.003490651415223739937 ) ) ;
#97208=VECTOR ( 'NONE', #104622, 1000.000000000000000 ) ;
#97209=EDGE_LOOP ( 'NONE', ( #85042, #35947 ) ) ;
#97210=FACE_BOUND ( 'NONE', #40529, .T. ) ;
#97211=DIRECTION ( 'NONE',  ( 0.000000000000000000, 1.000000000000000000, 0.000000000000000000 ) ) ;
#97212=ORIENTED_EDGE ( 'NONE', *, *, #66103, .F. ) ;
#97213=DIRECTION ( 'NONE',  ( -0.000000000000000000, -1.000000000000000000, -0.000000000000000000 ) ) ;
#97214=FACE_OUTER_BOUND ( 'NONE', #68169, .T. ) ;
#97215=ADVANCED_FACE ( 'NONE', ( #65218 ), #3569, .T. ) ;
#97216=VERTEX_POINT ( 'NONE', #116258 ) ;
#97217=CIRCLE ( 'NONE', #40815, 0.1000000000000002554 ) ;
#97218=EDGE_LOOP ( 'NONE', ( #74987, #96911 ) ) ;
#97219=AXIS2_PLACEMENT_3D ( 'NONE', #36584, #64086, #14948 ) ;
#97221=DIRECTION ( 'NONE',  ( -0.000000000000000000, -1.000000000000000000, -0.000000000000000000 ) ) ;
#97222=FACE_OUTER_BOUND ( 'NONE', #22679, .T. ) ;
#97223=DIRECTION ( 'NONE',  ( -0.000000000000000000, 1.000000000000000000, -0.000000000000000000 ) ) ;
#97224=FACE_BOUND ( 'NONE', #84125, .T. ) ;
#97225=VERTEX_POINT ( 'NONE', #4348 ) ;
#97226=CARTESIAN_POINT ( 'NONE',  ( 12.09999999999990550, 2.500000000000000000, 4.330127018922196314 ) ) ;
#97227=DIRECTION ( 'NONE',  ( 0.000000000000000000, 0.000000000000000000, 1.000000000000000000 ) ) ;
#97229=VECTOR ( 'NONE', #74219, 1000.000000000000000 ) ;
#97230=DIRECTION ( 'NONE',  ( -4.274815082592931898E-19, -0.9999939076577903929, -0.003490651415223739937 ) ) ;
#97231=ADVANCED_FACE ( 'NONE', ( #44299 ), #114282, .T. ) ;
#97232=DIRECTION ( 'NONE',  ( -4.274815082592931898E-19, -0.9999939076577903929, -0.003490651415223739937 ) ) ;
#97233=DIRECTION ( 'NONE',  ( -0.000000000000000000, -1.000000000000000000, -0.000000000000000000 ) ) ;
#97234=DIRECTION ( 'NONE',  ( 0.000000000000000000, -0.000000000000000000, 1.000000000000000000 ) ) ;
#97235=CARTESIAN_POINT ( 'NONE',  ( -4.200000000000025935, 2.500000000000000000, 4.330127018922196314 ) ) ;
#97236=ORIENTED_EDGE ( 'NONE', *, *, #92145, .F. ) ;
#97237=ORIENTED_EDGE ( 'NONE', *, *, #98744, .F. ) ;
#97238=ORIENTED_EDGE ( 'NONE', *, *, #16180, .T. ) ;
#97239=ORIENTED_EDGE ( 'NONE', *, *, #85771, .F. ) ;
#97240=ORIENTED_EDGE ( 'NONE', *, *, #92669, .T. ) ;
#97241=FACE_OUTER_BOUND ( 'NONE', #125245, .T. ) ;
#97242=LINE ( 'NONE', #47512, #80149 ) ;
#97243=ORIENTED_EDGE ( 'NONE', *, *, #22732, .T. ) ;
#97244=ADVANCED_FACE ( 'NONE', ( #29828 ), #59960, .T. ) ;
#97245=FACE_BOUND ( 'NONE', #43602, .T. ) ;
#97246=DIRECTION ( 'NONE',  ( 0.000000000000000000, 0.000000000000000000, 1.000000000000000000 ) ) ;
#97247=AXIS2_PLACEMENT_3D ( 'NONE', #84276, #122931, #31977 ) ;
#97248=DIRECTION ( 'NONE',  ( 0.000000000000000000, 0.000000000000000000, 1.000000000000000000 ) ) ;
#97249=AXIS2_PLACEMENT_3D ( 'NONE', #54649, #124705, #4253 ) ;
#97250=AXIS2_PLACEMENT_3D ( 'NONE', #39982, #109350, #68781 ) ;
#97251=CARTESIAN_POINT ( 'NONE',  ( -4.150000000000025224, 2.500000000000000000, 6.395190528383296602 ) ) ;
#97252=DIRECTION ( 'NONE',  ( 0.000000000000000000, 1.000000000000000000, 0.000000000000000000 ) ) ;
#97253=LINE ( 'NONE', #35137, #110198 ) ;
#97254=ORIENTED_EDGE ( 'NONE', *, *, #115753, .T. ) ;
#97255=DIRECTION ( 'NONE',  ( -0.000000000000000000, -1.000000000000000000, -0.000000000000000000 ) ) ;
#97256=VECTOR ( 'NONE', #95066, 1000.000000000000000 ) ;
#97257=ORIENTED_EDGE ( 'NONE', *, *, #104769, .F. ) ;
#97258=AXIS2_PLACEMENT_3D ( 'NONE', #36801, #28256, #76710 ) ;
#97259=ORIENTED_EDGE ( 'NONE', *, *, #54044, .F. ) ;
#97260=ORIENTED_EDGE ( 'NONE', *, *, #111179, .T. ) ;
#97261=DIRECTION ( 'NONE',  ( 0.000000000000000000, 0.000000000000000000, -1.000000000000000000 ) ) ;
#97262=CIRCLE ( 'NONE', #113994, 0.06509327318403745899 ) ;
#97263=CARTESIAN_POINT ( 'NONE',  ( -3.550000000000028688, 12.50000000000000000, 6.776507416713035248 ) ) ;
#97264=LINE ( 'NONE', #55415, #25856 ) ;
#97266=CARTESIAN_POINT ( 'NONE',  ( 3.677919667777222568, 2.499999999999998668, -8.999999999876376222 ) ) ;
#97267=AXIS2_PLACEMENT_3D ( 'NONE', #49523, #29871, #40350 ) ;
#97268=CIRCLE ( 'NONE', #32544, 0.06509327318403745899 ) ;
#97269=DIRECTION ( 'NONE',  ( 0.000000000000000000, 1.000000000000000000, 0.000000000000000000 ) ) ;
#97270=EDGE_CURVE ( 'NONE', #37520, #31054, #66256, .T. ) ;
#97271=DIRECTION ( 'NONE',  ( -0.000000000000000000, 1.000000000000000000, -0.000000000000000000 ) ) ;
#97273=PLANE ( 'NONE',  #103144 ) ;
#97275=AXIS2_PLACEMENT_3D ( 'NONE', #114708, #106195, #101842 ) ;
#97276=DIRECTION ( 'NONE',  ( 0.000000000000000000, -0.9999939076577903929, 0.003490651415223739937 ) ) ;
#97277=ORIENTED_EDGE ( 'NONE', *, *, #110931, .T. ) ;
#97278=CARTESIAN_POINT ( 'NONE',  ( -11.64999999999999680, 2.500000000000000000, 2.857883832488649301 ) ) ;
#97279=EDGE_CURVE ( 'NONE', #21310, #40453, #112242, .T. ) ;
#97280=ORIENTED_EDGE ( 'NONE', *, *, #94612, .F. ) ;
#97281=VERTEX_POINT ( 'NONE', #97910 ) ;
#97282=DIRECTION ( 'NONE',  ( 0.000000000000000000, -0.000000000000000000, 1.000000000000000000 ) ) ;
#97283=EDGE_CURVE ( 'NONE', #92671, #74675, #1409, .T. ) ;
#97284=CARTESIAN_POINT ( 'NONE',  ( -10.65000000000000213, 2.500000000000000000, 6.841600689897072485 ) ) ;
#97285=CARTESIAN_POINT ( 'NONE',  ( 3.149999999999946176, 12.50000000000000000, -1.753560074763288457 ) ) ;
#97286=ADVANCED_FACE ( 'NONE', ( #29200 ), #117526, .T. ) ;
#97287=EDGE_CURVE ( 'NONE', #74651, #84244, #72541, .T. ) ;
#97288=EDGE_CURVE ( 'NONE', #109488, #29207, #76732, .T. ) ;
#97289=AXIS2_PLACEMENT_3D ( 'NONE', #127677, #95010, #66809 ) ;
#97290=VERTEX_POINT ( 'NONE', #10188 ) ;
#97291=ORIENTED_EDGE ( 'NONE', *, *, #86145, .T. ) ;
#97292=CARTESIAN_POINT ( 'NONE',  ( 11.24999999999990763, 2.500000000000000000, 1.472243186433545459 ) ) ;
#97293=CARTESIAN_POINT ( 'NONE',  ( 11.64999999999990443, 2.500000000000000000, 2.857883832488649301 ) ) ;
#97294=ADVANCED_FACE ( 'NONE', ( #69093 ), #27887, .T. ) ;
#97295=CARTESIAN_POINT ( 'NONE',  ( -7.700000000000014388, 2.500000000000000000, -4.776537180435977525 ) ) ;
#97296=ORIENTED_EDGE ( 'NONE', *, *, #27611, .F. ) ;
#97297=ORIENTED_EDGE ( 'NONE', *, *, #123517, .T. ) ;
#97298=ADVANCED_FACE ( 'NONE', ( #27235 ), #93455, .T. ) ;
#97299=FACE_OUTER_BOUND ( 'NONE', #24532, .T. ) ;
#97300=AXIS2_PLACEMENT_3D ( 'NONE', #119962, #91144, #30314 ) ;
#97301=EDGE_CURVE ( 'NONE', #66020, #27914, #20295, .T. ) ;
#97302=AXIS2_PLACEMENT_3D ( 'NONE', #49321, #8071, #127224 ) ;
#97303=ORIENTED_EDGE ( 'NONE', *, *, #26542, .F. ) ;
#97304=DIRECTION ( 'NONE',  ( 0.000000000000000000, -0.000000000000000000, 1.000000000000000000 ) ) ;
#97305=AXIS2_PLACEMENT_3D ( 'NONE', #14148, #56642, #86102 ) ;
#97306=EDGE_CURVE ( 'NONE', #120320, #54255, #75004, .T. ) ;
#97307=EDGE_CURVE ( 'NONE', #30363, #98217, #18707, .T. ) ;
#97308=CARTESIAN_POINT ( 'NONE',  ( -2.700000000000030820, 2.500000000000000000, 0.3464101615137735735 ) ) ;
#97309=ORIENTED_EDGE ( 'NONE', *, *, #14338, .T. ) ;
#97310=DIRECTION ( 'NONE',  ( 0.000000000000000000, 0.000000000000000000, 1.000000000000000000 ) ) ;
#97311=DIRECTION ( 'NONE',  ( -0.000000000000000000, 1.000000000000000000, -0.000000000000000000 ) ) ;
#97312=DIRECTION ( 'NONE',  ( 0.000000000000000000, 0.000000000000000000, 1.000000000000000000 ) ) ;
#97313=DIRECTION ( 'NONE',  ( -4.274815082592931898E-19, -0.9999939076577903929, -0.003490651415223739937 ) ) ;
#97314=EDGE_CURVE ( 'NONE', #45883, #50211, #24825, .T. ) ;
#97315=ORIENTED_EDGE ( 'NONE', *, *, #43195, .F. ) ;
#97316=AXIS2_PLACEMENT_3D ( 'NONE', #88332, #1269, #18957 ) ;
#97317=CARTESIAN_POINT ( 'NONE',  ( 10.39999999999991154, 2.500000000000000000, 3.637306695894644726 ) ) ;
#97318=CONICAL_SURFACE ( 'NONE', #17887, 0.1000000000000002554, 0.003490658503988666988 ) ;
#97319=EDGE_LOOP ( 'NONE', ( #25443, #63113 ) ) ;
#97320=ORIENTED_EDGE ( 'NONE', *, *, #123175, .T. ) ;
#97321=FACE_OUTER_BOUND ( 'NONE', #5446, .T. ) ;
#97322=CARTESIAN_POINT ( 'NONE',  ( 9.799999999999915445, 2.500000000000000000, 4.083716857408421497 ) ) ;
#97323=DIRECTION ( 'NONE',  ( 0.000000000000000000, -0.9999939076577903929, 0.003490651415223739937 ) ) ;
#97324=DIRECTION ( 'NONE',  ( -4.274815082592931898E-19, -0.9999939076577903929, -0.003490651415223739937 ) ) ;
#97325=DIRECTION ( 'NONE',  ( 0.000000000000000000, -0.9999939076577903929, 0.003490651415223739937 ) ) ;
#97326=DIRECTION ( 'NONE',  ( 0.000000000000000000, 1.000000000000000000, 0.000000000000000000 ) ) ;
#97327=AXIS2_PLACEMENT_3D ( 'NONE', #3541, #33024, #2233 ) ;
#97328=CARTESIAN_POINT ( 'NONE',  ( 17.50982738792208693, 2.500000000000000000, -4.074750937467086942 ) ) ;
#97329=CARTESIAN_POINT ( 'NONE',  ( 6.249999999999967137, 2.500000000000000000, -2.165063509461101710 ) ) ;
#97330=LINE ( 'NONE', #56727, #23348 ) ;
#97331=FACE_OUTER_BOUND ( 'NONE', #127722, .T. ) ;
#97332=VERTEX_POINT ( 'NONE', #19342 ) ;
#97333=CARTESIAN_POINT ( 'NONE',  ( -13.09999999999999076, 2.500000000000000000, 4.083716857408421497 ) ) ;
#97334=DIRECTION ( 'NONE',  ( -4.274815082592931898E-19, -0.9999939076577903929, -0.003490651415223739937 ) ) ;
#97335=CARTESIAN_POINT ( 'NONE',  ( 4.149999999999941735, 2.500000000000000000, -1.472243186433550122 ) ) ;
#97336=AXIS2_PLACEMENT_3D ( 'NONE', #126933, #119041, #97462 ) ;
#97337=CARTESIAN_POINT ( 'NONE',  ( -2.500000000000032419, 12.50000000000000000, -3.637306695894650055 ) ) ;
#97338=DIRECTION ( 'NONE',  ( 0.000000000000000000, 0.000000000000000000, 1.000000000000000000 ) ) ;
#97339=VERTEX_POINT ( 'NONE', #107738 ) ;
#97340=DIRECTION ( 'NONE',  ( 0.000000000000000000, 0.000000000000000000, 1.000000000000000000 ) ) ;
#97341=ADVANCED_FACE ( 'NONE', ( #18057 ), #77059, .T. ) ;
#97342=CONICAL_SURFACE ( 'NONE', #34672, 0.09999999999999982514, 0.003490658503988666988 ) ;
#97343=CONICAL_SURFACE ( 'NONE', #116121, 0.1000000000000000472, 0.003490658503988666988 ) ;
#97344=EDGE_CURVE ( 'NONE', #34729, #45963, #48176, .T. ) ;
#97345=FACE_OUTER_BOUND ( 'NONE', #44786, .T. ) ;
#97346=DIRECTION ( 'NONE',  ( 0.000000000000000000, -0.9999939076577903929, 0.003490651415223739937 ) ) ;
#97347=ORIENTED_EDGE ( 'NONE', *, *, #27347, .F. ) ;
#97348=ORIENTED_EDGE ( 'NONE', *, *, #45590, .T. ) ;
#97349=CONICAL_SURFACE ( 'NONE', #67816, 0.1000000000000000056, 0.003490658503988666988 ) ;
#97350=ADVANCED_FACE ( 'NONE', ( #48834 ), #33157, .T. ) ;
#97351=EDGE_LOOP ( 'NONE', ( #51258, #94429, #6311, #63576 ) ) ;
#97352=ORIENTED_EDGE ( 'NONE', *, *, #100325, .F. ) ;
#97353=EDGE_LOOP ( 'NONE', ( #122260, #46902 ) ) ;
#97354=DIRECTION ( 'NONE',  ( 0.000000000000000000, 0.000000000000000000, 1.000000000000000000 ) ) ;
#97355=CARTESIAN_POINT ( 'NONE',  ( 3.749999999999975131, 12.50000000000000000, 6.495190528383297135 ) ) ;
#97356=LINE ( 'NONE', #107165, #83866 ) ;
#97357=VECTOR ( 'NONE', #76249, 1000.000000000000000 ) ;
#97358=DIRECTION ( 'NONE',  ( 0.000000000000000000, 0.000000000000000000, 1.000000000000000000 ) ) ;
#97359=CIRCLE ( 'NONE', #15878, 0.06509327318403745899 ) ;
#97360=ORIENTED_EDGE ( 'NONE', *, *, #11465, .F. ) ;
#97361=CIRCLE ( 'NONE', #43018, 0.1000000000000000472 ) ;
#97362=DIRECTION ( 'NONE',  ( -0.000000000000000000, -1.000000000000000000, -0.000000000000000000 ) ) ;
#97363=CIRCLE ( 'NONE', #55327, 0.06509327318403745899 ) ;
#97364=VERTEX_POINT ( 'NONE', #61879 ) ;
#97365=CARTESIAN_POINT ( 'NONE',  ( 32.27111852109496226, -3.178312372603624425, -3.140919221371700321 ) ) ;
#97366=CARTESIAN_POINT ( 'NONE',  ( 12.30568799110296396, -2.500000000000000000, -7.490555764796996918 ) ) ;
#97368=DIRECTION ( 'NONE',  ( 0.000000000000000000, 1.000000000000000000, 0.000000000000000000 ) ) ;
#97369=CARTESIAN_POINT ( 'NONE',  ( 1.049999999999954525, 2.500000000000000000, 1.818653347947321475 ) ) ;
#97370=ORIENTED_EDGE ( 'NONE', *, *, #16029, .F. ) ;
#97371=EDGE_LOOP ( 'NONE', ( #6796, #117552, #15051, #3771 ) ) ;
#97372=VERTEX_POINT ( 'NONE', #95036 ) ;
#97373=EDGE_LOOP ( 'NONE', ( #72685, #58447, #86839, #91996 ) ) ;
#97374=FACE_OUTER_BOUND ( 'NONE', #122893, .T. ) ;
#97375=DIRECTION ( 'NONE',  ( 0.000000000000000000, 1.000000000000000000, 0.000000000000000000 ) ) ;
#97376=CARTESIAN_POINT ( 'NONE',  ( -4.350000000000023626, 2.500000000000000000, -2.611473670974877592 ) ) ;
#97377=FACE_BOUND ( 'NONE', #112748, .T. ) ;
#97378=DIRECTION ( 'NONE',  ( -4.274815082592931898E-19, -0.9999939076577903929, -0.003490651415223739937 ) ) ;
#97379=DIRECTION ( 'NONE',  ( 0.000000000000000000, -1.000000000000000000, 0.000000000000000000 ) ) ;
#97380=DIRECTION ( 'NONE',  ( -4.274815082592931898E-19, -0.9999939076577903929, -0.003490651415223739937 ) ) ;
#97381=DIRECTION ( 'NONE',  ( 0.000000000000000000, 0.000000000000000000, 1.000000000000000000 ) ) ;
#97382=EDGE_CURVE ( 'NONE', #68683, #6418, #100049, .T. ) ;
#97384=DIRECTION ( 'NONE',  ( -0.000000000000000000, -1.000000000000000000, -0.000000000000000000 ) ) ;
#97385=DIRECTION ( 'NONE',  ( 0.000000000000000000, 0.000000000000000000, -1.000000000000000000 ) ) ;
#97386=CIRCLE ( 'NONE', #43047, 0.06509327318403745899 ) ;
#97387=VECTOR ( 'NONE', #6730, 1000.000000000000000 ) ;
#97388=DIRECTION ( 'NONE',  ( 0.000000000000000000, 0.000000000000000000, 1.000000000000000000 ) ) ;
#97389=AXIS2_PLACEMENT_3D ( 'NONE', #49120, #109304, #51054 ) ;
#97390=VERTEX_POINT ( 'NONE', #70395 ) ;
#97391=EDGE_LOOP ( 'NONE', ( #28050, #128579 ) ) ;
#97392=ORIENTED_EDGE ( 'NONE', *, *, #5105, .T. ) ;
#97393=ORIENTED_EDGE ( 'NONE', *, *, #54347, .F. ) ;
#97394=EDGE_CURVE ( 'NONE', #103978, #125076, #4683, .T. ) ;
#97395=CARTESIAN_POINT ( 'NONE',  ( -8.150000000000009237, 2.500000000000000000, 6.841600689897072485 ) ) ;
#97396=ADVANCED_FACE ( 'NONE', ( #52053 ), #20636, .T. ) ;
#97397=FACE_BOUND ( 'NONE', #123685, .T. ) ;
#97398=CARTESIAN_POINT ( 'NONE',  ( 11.04999999999990656, 2.500000000000000000, 2.411473670974873862 ) ) ;
#97400=CONICAL_SURFACE ( 'NONE', #34738, 0.1000000000000002554, 0.003490658503988666988 ) ;
#97401=CIRCLE ( 'NONE', #9583, 0.06509327318403745899 ) ;
#97402=ORIENTED_EDGE ( 'NONE', *, *, #125004, .T. ) ;
#97403=DIRECTION ( 'NONE',  ( -4.274815082592931898E-19, -0.9999939076577903929, -0.003490651415223739937 ) ) ;
#97404=EDGE_CURVE ( 'NONE', #115977, #13480, #106302, .T. ) ;
#97405=DIRECTION ( 'NONE',  ( 0.000000000000000000, -0.000000000000000000, 1.000000000000000000 ) ) ;
#97407=ORIENTED_EDGE ( 'NONE', *, *, #18905, .T. ) ;
#97409=DIRECTION ( 'NONE',  ( -0.000000000000000000, 1.000000000000000000, -0.000000000000000000 ) ) ;
#97410=AXIS2_PLACEMENT_3D ( 'NONE', #2107, #23055, #81964 ) ;
#97411=ORIENTED_EDGE ( 'NONE', *, *, #47959, .F. ) ;
#97412=CARTESIAN_POINT ( 'NONE',  ( 6.649999999999931966, 2.500000000000000000, -5.802370205355749988 ) ) ;
#97413=DIRECTION ( 'NONE',  ( 0.000000000000000000, -0.000000000000000000, 1.000000000000000000 ) ) ;
#97414=ORIENTED_EDGE ( 'NONE', *, *, #31860, .F. ) ;
#97415=CARTESIAN_POINT ( 'NONE',  ( 1.649999999999951950, 12.50000000000000000, -7.188010851410854052 ) ) ;
#97416=PLANE ( 'NONE',  #66509 ) ;
#97417=VERTEX_POINT ( 'NONE', #32434 ) ;
#97418=FACE_OUTER_BOUND ( 'NONE', #68435, .T. ) ;
#97419=ORIENTED_EDGE ( 'NONE', *, *, #22365, .F. ) ;
#97420=ORIENTED_EDGE ( 'NONE', *, *, #44709, .F. ) ;
#97421=CARTESIAN_POINT ( 'NONE',  ( -11.64999999999999680, 12.50000000000000000, 2.922977105672686982 ) ) ;
#97422=VERTEX_POINT ( 'NONE', #20657 ) ;
#97423=DIRECTION ( 'NONE',  ( 0.000000000000000000, 1.000000000000000000, 0.000000000000000000 ) ) ;
#97424=FACE_BOUND ( 'NONE', #42522, .T. ) ;
#97425=EDGE_CURVE ( 'NONE', #93012, #82725, #26884, .T. ) ;
#97426=CIRCLE ( 'NONE', #82873, 0.06509327318403745899 ) ;
#97427=ORIENTED_EDGE ( 'NONE', *, *, #76194, .T. ) ;
#97428=AXIS2_PLACEMENT_3D ( 'NONE', #96, #78016, #97013 ) ;
#97430=EDGE_LOOP ( 'NONE', ( #62063, #75335, #119105, #122412 ) ) ;
#97432=CARTESIAN_POINT ( 'NONE',  ( 9.999999999999912959, 12.50000000000000000, 3.637306695894644726 ) ) ;
#97433=CARTESIAN_POINT ( 'NONE',  ( -4.550000000000022915, 2.500000000000000000, 6.495190528383297135 ) ) ;
#97434=CARTESIAN_POINT ( 'NONE',  ( 4.149999999999939959, 12.50000000000000000, -6.430097255199264339 ) ) ;
#97435=ADVANCED_FACE ( 'NONE', ( #91966 ), #104248, .T. ) ;
#97436=CARTESIAN_POINT ( 'NONE',  ( 3.749999999999978684, 2.500000000000000000, -2.165063509461101710 ) ) ;
#97437=EDGE_CURVE ( 'NONE', #106593, #85023, #12194, .T. ) ;
#97438=VECTOR ( 'NONE', #116812, 1000.000000000000000 ) ;
#97439=CONICAL_SURFACE ( 'NONE', #13801, 0.1000000000000000472, 0.003490658503988666988 ) ;
#97441=ORIENTED_EDGE ( 'NONE', *, *, #67031, .T. ) ;
#97442=DIRECTION ( 'NONE',  ( 0.000000000000000000, 0.000000000000000000, 1.000000000000000000 ) ) ;
#97443=CARTESIAN_POINT ( 'NONE',  ( 6.449999999999931788, 12.50000000000000000, -6.213873640053564351 ) ) ;
#97444=EDGE_CURVE ( 'NONE', #113589, #61474, #37361, .T. ) ;
#97445=CARTESIAN_POINT ( 'NONE',  ( 3.549999999999944755, 2.500000000000000000, -2.611473670974877592 ) ) ;
#97446=VERTEX_POINT ( 'NONE', #12107 ) ;
#97448=EDGE_CURVE ( 'NONE', #55495, #19791, #16385, .T. ) ;
#97450=ADVANCED_FACE ( 'NONE', ( #100490 ), #110505, .T. ) ;
#97451=CARTESIAN_POINT ( 'NONE',  ( 5.849999999999933920, 2.500000000000000000, -2.165063509461101710 ) ) ;
#97452=AXIS2_PLACEMENT_3D ( 'NONE', #117264, #75427, #67526 ) ;
#97453=VECTOR ( 'NONE', #79992, 1000.000000000000000 ) ;
#97454=DIRECTION ( 'NONE',  ( -0.000000000000000000, -1.000000000000000000, -0.000000000000000000 ) ) ;
#97455=LINE ( 'NONE', #110961, #66531 ) ;
#97456=AXIS2_PLACEMENT_3D ( 'NONE', #87776, #127712, #126442 ) ;
#97458=EDGE_CURVE ( 'NONE', #66944, #121198, #121416, .T. ) ;
#97459=DIRECTION ( 'NONE',  ( 0.000000000000000000, 0.000000000000000000, -1.000000000000000000 ) ) ;
#97460=DIRECTION ( 'NONE',  ( -0.000000000000000000, -1.000000000000000000, -0.000000000000000000 ) ) ;
#97461=CARTESIAN_POINT ( 'NONE',  ( 15.39999999999989200, 2.500000000000000000, 0.7928203230275495672 ) ) ;
#97462=DIRECTION ( 'NONE',  ( 0.000000000000000000, 0.000000000000000000, 1.000000000000000000 ) ) ;
#97463=DIRECTION ( 'NONE',  ( 0.000000000000000000, -0.9999939076577903929, 0.003490651415223739937 ) ) ;
#97464=EDGE_CURVE ( 'NONE', #129286, #118274, #64910, .T. ) ;
#97465=DIRECTION ( 'NONE',  ( 0.000000000000000000, 0.000000000000000000, 1.000000000000000000 ) ) ;
#97466=EDGE_CURVE ( 'NONE', #91316, #90767, #51938, .T. ) ;
#97467=VERTEX_POINT ( 'NONE', #120142 ) ;
#97468=ORIENTED_EDGE ( 'NONE', *, *, #17448, .T. ) ;
#97469=CARTESIAN_POINT ( 'NONE',  ( 6.649999999999931077, 12.50000000000000000, -6.560283801567339701 ) ) ;
#97470=VERTEX_POINT ( 'NONE', #74750 ) ;
#97471=EDGE_LOOP ( 'NONE', ( #121239, #106894 ) ) ;
#97472=CARTESIAN_POINT ( 'NONE',  ( 11.64999999999990266, 12.50000000000000000, -6.430097255199264339 ) ) ;
#97473=DIRECTION ( 'NONE',  ( 0.000000000000000000, 0.000000000000000000, -1.000000000000000000 ) ) ;
#97474=CIRCLE ( 'NONE', #39018, 0.06509327318403745899 ) ;
#97475=CARTESIAN_POINT ( 'NONE',  ( -5.400000000000023448, 12.50000000000000000, -5.088040615133791356 ) ) ;
#97476=CARTESIAN_POINT ( 'NONE',  ( -8.550000000000013145, 2.500000000000000000, 2.611473670974873151 ) ) ;
#97477=DIRECTION ( 'NONE',  ( 0.000000000000000000, 1.000000000000000000, 0.000000000000000000 ) ) ;
#97478=DIRECTION ( 'NONE',  ( 0.000000000000000000, 0.000000000000000000, 1.000000000000000000 ) ) ;
#97479=CIRCLE ( 'NONE', #87010, 0.09999999999999982514 ) ;
#97480=DIRECTION ( 'NONE',  ( -0.000000000000000000, -1.000000000000000000, -0.000000000000000000 ) ) ;
#97481=VERTEX_POINT ( 'NONE', #114659 ) ;
#97482=DIRECTION ( 'NONE',  ( 0.000000000000000000, 1.000000000000000000, 0.000000000000000000 ) ) ;
#97483=CIRCLE ( 'NONE', #124681, 0.1000000000000002554 ) ;
#97484=CIRCLE ( 'NONE', #28536, 0.09999999999999982514 ) ;
#97485=VECTOR ( 'NONE', #27678, 1000.000000000000000 ) ;
#97486=CARTESIAN_POINT ( 'NONE',  ( -10.65000000000000391, 2.500000000000000000, -2.511473670974873951 ) ) ;
#97488=VECTOR ( 'NONE', #7066, 1000.000000000000000 ) ;
#97489=ORIENTED_EDGE ( 'NONE', *, *, #59480, .F. ) ;
#97490=EDGE_LOOP ( 'NONE', ( #30458, #116483, #46311, #50284 ) ) ;
#97491=ORIENTED_EDGE ( 'NONE', *, *, #67109, .T. ) ;
#97492=DIRECTION ( 'NONE',  ( 0.000000000000000000, 1.000000000000000000, 0.000000000000000000 ) ) ;
#97493=DIRECTION ( 'NONE',  ( 0.000000000000000000, 0.000000000000000000, 1.000000000000000000 ) ) ;
#97494=AXIS2_PLACEMENT_3D ( 'NONE', #11572, #51513, #22061 ) ;
#97495=ORIENTED_EDGE ( 'NONE', *, *, #40082, .F. ) ;
#97496=DIRECTION ( 'NONE',  ( -0.000000000000000000, 1.000000000000000000, -0.000000000000000000 ) ) ;
#97497=EDGE_CURVE ( 'NONE', #43212, #124362, #8706, .T. ) ;
#97498=CARTESIAN_POINT ( 'NONE',  ( -4.350000000000027178, 12.50000000000000000, -6.841600689897077814 ) ) ;
#97499=AXIS2_PLACEMENT_3D ( 'NONE', #61407, #91493, #1813 ) ;
#97500=AXIS2_PLACEMENT_3D ( 'NONE', #6589, #17052, #27537 ) ;
#97501=EDGE_CURVE ( 'NONE', #61453, #36022, #45675, .T. ) ;
#97502=DIRECTION ( 'NONE',  ( 0.000000000000000000, 1.000000000000000000, 0.000000000000000000 ) ) ;
#97503=ORIENTED_EDGE ( 'NONE', *, *, #61971, .T. ) ;
#97504=DIRECTION ( 'NONE',  ( 0.000000000000000000, -0.000000000000000000, 1.000000000000000000 ) ) ;
#97505=CARTESIAN_POINT ( 'NONE',  ( 2.049999999999950084, 2.500000000000000000, 2.165063509461097713 ) ) ;
#97506=ORIENTED_EDGE ( 'NONE', *, *, #125339, .F. ) ;
#97507=ORIENTED_EDGE ( 'NONE', *, *, #41042, .F. ) ;
#97508=ORIENTED_EDGE ( 'NONE', *, *, #58877, .F. ) ;
#97509=DIRECTION ( 'NONE',  ( 0.000000000000000000, -0.000000000000000000, 1.000000000000000000 ) ) ;
#97510=DIRECTION ( 'NONE',  ( -0.000000000000000000, 1.000000000000000000, -0.000000000000000000 ) ) ;
#97511=VERTEX_POINT ( 'NONE', #106766 ) ;
#97512=FACE_OUTER_BOUND ( 'NONE', #89176, .T. ) ;
#97513=CARTESIAN_POINT ( 'NONE',  ( 11.04999999999991189, 12.50000000000000000, 6.083687093685483660 ) ) ;
#97514=PLANE ( 'NONE',  #35807 ) ;
#97515=CARTESIAN_POINT ( 'NONE',  ( -1.450000000000035483, 12.50000000000000000, 6.213873640053559022 ) ) ;
#97516=VERTEX_POINT ( 'NONE', #27551 ) ;
#97517=CONICAL_SURFACE ( 'NONE', #53618, 0.1000000000000002554, 0.003490658503988666988 ) ;
#97518=FACE_OUTER_BOUND ( 'NONE', #17204, .T. ) ;
#97519=AXIS2_PLACEMENT_3D ( 'NONE', #52278, #129575, #10408 ) ;
#97520=EDGE_LOOP ( 'NONE', ( #95634, #39601, #22141, #129366 ) ) ;
#97521=VERTEX_POINT ( 'NONE', #96952 ) ;
#97522=DIRECTION ( 'NONE',  ( 0.000000000000000000, 1.000000000000000000, 0.000000000000000000 ) ) ;
#97523=CARTESIAN_POINT ( 'NONE',  ( 8.149999999999923972, 12.50000000000000000, -6.841600689897077814 ) ) ;
#97524=FACE_BOUND ( 'NONE', #59944, .T. ) ;
#97526=DIRECTION ( 'NONE',  ( 0.000000000000000000, 1.000000000000000000, 0.000000000000000000 ) ) ;
#97527=CIRCLE ( 'NONE', #36912, 0.06509327318403745899 ) ;
#97528=DIRECTION ( 'NONE',  ( -0.000000000000000000, 1.000000000000000000, -0.000000000000000000 ) ) ;
#97529=EDGE_CURVE ( 'NONE', #106540, #17110, #87503, .T. ) ;
#97530=ORIENTED_EDGE ( 'NONE', *, *, #30655, .F. ) ;
#97531=DIRECTION ( 'NONE',  ( -0.000000000000000000, 1.000000000000000000, -0.000000000000000000 ) ) ;
#97532=DIRECTION ( 'NONE',  ( -4.274815082592931898E-19, -0.9999939076577903929, -0.003490651415223739937 ) ) ;
#97533=DIRECTION ( 'NONE',  ( 0.000000000000000000, 1.000000000000000000, 0.000000000000000000 ) ) ;
#97534=DIRECTION ( 'NONE',  ( -0.000000000000000000, -1.000000000000000000, -0.000000000000000000 ) ) ;
#97535=ORIENTED_EDGE ( 'NONE', *, *, #111289, .T. ) ;
#97536=CONICAL_SURFACE ( 'NONE', #41135, 0.1000000000000000472, 0.003490658503988666988 ) ;
#97537=AXIS2_PLACEMENT_3D ( 'NONE', #21064, #61657, #112039 ) ;
#97538=ADVANCED_FACE ( 'NONE', ( #46556 ), #66582, .T. ) ;
#97539=CARTESIAN_POINT ( 'NONE',  ( -1.900000000000034106, 2.500000000000000000, -3.983716857408426293 ) ) ;
#97540=AXIS2_PLACEMENT_3D ( 'NONE', #34698, #12442, #73955 ) ;
#97541=CARTESIAN_POINT ( 'NONE',  ( 6.699999999999930012, 2.500000000000000000, -4.430127018922202176 ) ) ;
#97542=ORIENTED_EDGE ( 'NONE', *, *, #48710, .T. ) ;
#97544=EDGE_CURVE ( 'NONE', #18257, #7901, #85371, .T. ) ;
#97545=CARTESIAN_POINT ( 'NONE',  ( 3.149999999999942624, 2.500000000000000000, 6.248780366869521430 ) ) ;
#97546=DIRECTION ( 'NONE',  ( 0.000000000000000000, 0.000000000000000000, 1.000000000000000000 ) ) ;
#97547=EDGE_CURVE ( 'NONE', #122621, #129104, #75372, .T. ) ;
#97548=FACE_BOUND ( 'NONE', #43980, .T. ) ;
#97549=CARTESIAN_POINT ( 'NONE',  ( -15.19999999999998153, 2.500000000000000000, -0.3464101615137759604 ) ) ;
#97550=VERTEX_POINT ( 'NONE', #47224 ) ;
#97551=FACE_OUTER_BOUND ( 'NONE', #2803, .T. ) ;
#97552=EDGE_CURVE ( 'NONE', #12366, #51199, #62407, .T. ) ;
#97553=ORIENTED_EDGE ( 'NONE', *, *, #88399, .T. ) ;
#97554=ORIENTED_EDGE ( 'NONE', *, *, #37325, .F. ) ;
#97555=DIRECTION ( 'NONE',  ( 0.000000000000000000, -0.000000000000000000, 1.000000000000000000 ) ) ;
#97556=ADVANCED_FACE ( 'NONE', ( #87130 ), #120972, .T. ) ;
#97558=AXIS2_PLACEMENT_3D ( 'NONE', #103876, #26603, #126078 ) ;
#97559=ORIENTED_EDGE ( 'NONE', *, *, #55020, .F. ) ;
#97560=CARTESIAN_POINT ( 'NONE',  ( 1.249999999999953815, 2.500000000000000000, 1.372243186433545370 ) ) ;
#97561=AXIS2_PLACEMENT_3D ( 'NONE', #837, #123202, #30965 ) ;
#97563=AXIS2_PLACEMENT_3D ( 'NONE', #86074, #115539, #127329 ) ;
#97564=CARTESIAN_POINT ( 'NONE',  ( -10.65000000000000213, 12.50000000000000000, 1.818653347947321475 ) ) ;
#97565=DIRECTION ( 'NONE',  ( 0.000000000000000000, 0.000000000000000000, 1.000000000000000000 ) ) ;
#97566=AXIS2_PLACEMENT_3D ( 'NONE', #71166, #10319, #69220 ) ;
#97567=CIRCLE ( 'NONE', #72552, 0.06509327318403745899 ) ;
#97568=ORIENTED_EDGE ( 'NONE', *, *, #93171, .F. ) ;
#97569=CIRCLE ( 'NONE', #70394, 0.06509327318403745899 ) ;
#97570=LINE ( 'NONE', #77289, #39276 ) ;
#97571=DIRECTION ( 'NONE',  ( 0.000000000000000000, -0.9999939076577903929, 0.003490651415223739937 ) ) ;
#97572=DIRECTION ( 'NONE',  ( 0.000000000000000000, 0.000000000000000000, -1.000000000000000000 ) ) ;
#97573=VERTEX_POINT ( 'NONE', #37409 ) ;
#97574=CARTESIAN_POINT ( 'NONE',  ( 87.50000000000001421, 3.975344334345554120, -6.360552532166837914 ) ) ;
#97575=ORIENTED_EDGE ( 'NONE', *, *, #100636, .T. ) ;
#97576=CIRCLE ( 'NONE', #28641, 0.1000000000000002554 ) ;
#97577=DIRECTION ( 'NONE',  ( 0.000000000000000000, 0.000000000000000000, -1.000000000000000000 ) ) ;
#97578=AXIS2_PLACEMENT_3D ( 'NONE', #18815, #58752, #48940 ) ;
#97579=ORIENTED_EDGE ( 'NONE', *, *, #12192, .F. ) ;
#97580=DIRECTION ( 'NONE',  ( 0.000000000000000000, 0.000000000000000000, 1.000000000000000000 ) ) ;
#97581=CARTESIAN_POINT ( 'NONE',  ( 17.50000000000000000, -2.500000000000000000, -0.3333333333333280413 ) ) ;
#97582=EDGE_CURVE ( 'NONE', #27222, #32827, #102099, .T. ) ;
#97583=CARTESIAN_POINT ( 'NONE',  ( 10.44999999999991402, 2.500000000000000000, -2.265063509461101798 ) ) ;
#97584=CIRCLE ( 'NONE', #32858, 0.09999999999999982514 ) ;
#97585=AXIS2_PLACEMENT_3D ( 'NONE', #67443, #70533, #27532 ) ;
#97586=CARTESIAN_POINT ( 'NONE',  ( -14.14999999999998614, 2.500000000000000000, -2.957883832488651610 ) ) ;
#97587=EDGE_LOOP ( 'NONE', ( #107338, #87495, #56736, #8466 ) ) ;
#97588=CARTESIAN_POINT ( 'NONE',  ( -7.950000000000012612, 2.500000000000000000, -2.265063509461101798 ) ) ;
#97589=CARTESIAN_POINT ( 'NONE',  ( -4.600000000000028066, 12.50000000000000000, -5.022947341949754119 ) ) ;
#97592=ADVANCED_FACE ( 'NONE', ( #26934 ), #114701, .T. ) ;
#97593=DIRECTION ( 'NONE',  ( 0.000000000000000000, -0.000000000000000000, 1.000000000000000000 ) ) ;
#97594=ADVANCED_FACE ( 'NONE', ( #125137 ), #77317, .T. ) ;
#97595=ORIENTED_EDGE ( 'NONE', *, *, #29076, .F. ) ;
#97596=ORIENTED_EDGE ( 'NONE', *, *, #25472, .F. ) ;
#97597=DIRECTION ( 'NONE',  ( 0.000000000000000000, 1.000000000000000000, 0.000000000000000000 ) ) ;
#97598=VERTEX_POINT ( 'NONE', #96301 ) ;
#97599=DIRECTION ( 'NONE',  ( 0.000000000000000000, 0.000000000000000000, 1.000000000000000000 ) ) ;
#97600=EDGE_CURVE ( 'NONE', #85528, #42572, #15807, .T. ) ;
#97601=ORIENTED_EDGE ( 'NONE', *, *, #24851, .F. ) ;
#97602=ORIENTED_EDGE ( 'NONE', *, *, #54293, .T. ) ;
#97603=VERTEX_POINT ( 'NONE', #66840 ) ;
#97604=EDGE_CURVE ( 'NONE', #4802, #69367, #18472, .T. ) ;
#97605=AXIS2_PLACEMENT_3D ( 'NONE', #35784, #115613, #126081 ) ;
#97606=DIRECTION ( 'NONE',  ( 0.000000000000000000, 1.000000000000000000, 0.000000000000000000 ) ) ;
#97607=EDGE_CURVE ( 'NONE', #46462, #3084, #58289, .T. ) ;
#97608=CARTESIAN_POINT ( 'NONE',  ( 11.64999999999990621, 2.500000000000000000, 6.595190528383296780 ) ) ;
#97609=DIRECTION ( 'NONE',  ( 0.000000000000000000, 0.000000000000000000, 1.000000000000000000 ) ) ;
#97610=ADVANCED_FACE ( 'NONE', ( #108063 ), #67469, .T. ) ;
#97611=FACE_OUTER_BOUND ( 'NONE', #121146, .T. ) ;
#97612=DIRECTION ( 'NONE',  ( 0.000000000000000000, 1.000000000000000000, 0.000000000000000000 ) ) ;
#97613=DIRECTION ( 'NONE',  ( 0.000000000000000000, 0.000000000000000000, 1.000000000000000000 ) ) ;
#97614=CARTESIAN_POINT ( 'NONE',  ( -1.250000000000037970, 2.500000000000000000, 7.188010851410848723 ) ) ;
#97615=ORIENTED_EDGE ( 'NONE', *, *, #65533, .T. ) ;
#97616=CARTESIAN_POINT ( 'NONE',  ( 0.4499999999999573785, 2.500000000000000000, -6.495190528383302464 ) ) ;
#97617=EDGE_CURVE ( 'NONE', #9937, #56654, #17740, .T. ) ;
#97618=ORIENTED_EDGE ( 'NONE', *, *, #42178, .T. ) ;
#97619=EDGE_CURVE ( 'NONE', #7894, #70834, #47874, .T. ) ;
#97620=AXIS2_PLACEMENT_3D ( 'NONE', #95513, #45777, #122404 ) ;
#97621=EDGE_LOOP ( 'NONE', ( #58735, #83021, #7334, #36162 ) ) ;
#97622=EDGE_LOOP ( 'NONE', ( #24793, #93808 ) ) ;
#97623=ORIENTED_EDGE ( 'NONE', *, *, #80856, .T. ) ;
#97625=CARTESIAN_POINT ( 'NONE',  ( 7.699999999999923794, 12.50000000000000000, -0.2813168883297409439 ) ) ;
#97626=ORIENTED_EDGE ( 'NONE', *, *, #54533, .F. ) ;
#97627=VERTEX_POINT ( 'NONE', #58343 ) ;
#97628=CIRCLE ( 'NONE', #118551, 0.1000000000000002554 ) ;
#97629=CIRCLE ( 'NONE', #55853, 0.06509327318403745899 ) ;
#97630=DIRECTION ( 'NONE',  ( 0.000000000000000000, 0.000000000000000000, 1.000000000000000000 ) ) ;
#97631=DIRECTION ( 'NONE',  ( 0.000000000000000000, 1.000000000000000000, 0.000000000000000000 ) ) ;
#97632=CARTESIAN_POINT ( 'NONE',  ( 8.349999999999923261, 12.50000000000000000, -6.495190528383302464 ) ) ;
#97633=FACE_OUTER_BOUND ( 'NONE', #56530, .T. ) ;
#97634=DIRECTION ( 'NONE',  ( -0.000000000000000000, -1.000000000000000000, -0.000000000000000000 ) ) ;
#97635=EDGE_LOOP ( 'NONE', ( #70058, #25236, #26384, #43069 ) ) ;
#97636=CARTESIAN_POINT ( 'NONE',  ( -6.450000000000014388, 12.50000000000000000, 6.148780366869520897 ) ) ;
#97637=VECTOR ( 'NONE', #20715, 1000.000000000000000 ) ;
#97638=AXIS2_PLACEMENT_3D ( 'NONE', #107366, #7214, #127651 ) ;
#97639=ORIENTED_EDGE ( 'NONE', *, *, #85436, .F. ) ;
#97640=CARTESIAN_POINT ( 'NONE',  ( -8.550000000000009592, 12.50000000000000000, 6.841600689897072485 ) ) ;
#97641=AXIS2_PLACEMENT_3D ( 'NONE', #34326, #74231, #4178 ) ;
#97642=EDGE_LOOP ( 'NONE', ( #32906, #107695, #107333, #57087 ) ) ;
#97643=DIRECTION ( 'NONE',  ( -0.000000000000000000, -1.000000000000000000, -0.000000000000000000 ) ) ;
#97644=ORIENTED_EDGE ( 'NONE', *, *, #33156, .T. ) ;
#97645=VERTEX_POINT ( 'NONE', #79269 ) ;
#97646=CARTESIAN_POINT ( 'NONE',  ( -7.900000000000011013, 2.500000000000000000, 4.430127018922196847 ) ) ;
#97647=LINE ( 'NONE', #59687, #48558 ) ;
#97648=FACE_OUTER_BOUND ( 'NONE', #58345, .T. ) ;
#97649=ADVANCED_FACE ( 'NONE', ( #20336 ), #51100, .T. ) ;
#97650=LINE ( 'NONE', #98943, #69807 ) ;
#97651=CARTESIAN_POINT ( 'NONE',  ( -1.850000000000033396, 12.50000000000000000, -6.148780366869526226 ) ) ;
#97652=EDGE_LOOP ( 'NONE', ( #7820, #110640 ) ) ;
#97653=DIRECTION ( 'NONE',  ( 0.000000000000000000, 0.000000000000000000, 1.000000000000000000 ) ) ;
#97654=CARTESIAN_POINT ( 'NONE',  ( 10.44999999999991402, 2.500000000000000000, 6.595190528383296780 ) ) ;
#97655=CARTESIAN_POINT ( 'NONE',  ( -13.14999999999999147, 2.500000000000000000, 1.818653347947325472 ) ) ;
#97656=DIRECTION ( 'NONE',  ( 0.000000000000000000, 1.000000000000000000, 0.000000000000000000 ) ) ;
#97657=CIRCLE ( 'NONE', #47493, 0.06509327318403745899 ) ;
#97658=DIRECTION ( 'NONE',  ( 0.000000000000000000, -0.000000000000000000, 1.000000000000000000 ) ) ;
#97659=EDGE_CURVE ( 'NONE', #43021, #87479, #128834, .T. ) ;
#97660=ORIENTED_EDGE ( 'NONE', *, *, #52884, .T. ) ;
#97661=AXIS2_PLACEMENT_3D ( 'NONE', #61815, #81447, #72912 ) ;
#97663=CARTESIAN_POINT ( 'NONE',  ( -11.84999999999999787, 2.500000000000000000, -6.148780366869522673 ) ) ;
#97664=VECTOR ( 'NONE', #124633, 1000.000000000000000 ) ;
#97665=ORIENTED_EDGE ( 'NONE', *, *, #120950, .F. ) ;
#97666=AXIS2_PLACEMENT_3D ( 'NONE', #68433, #110302, #20645 ) ;
#97667=DIRECTION ( 'NONE',  ( 0.000000000000000000, 1.000000000000000000, 0.000000000000000000 ) ) ;
#97668=DIRECTION ( 'NONE',  ( 0.000000000000000000, -0.000000000000000000, 1.000000000000000000 ) ) ;
#97669=CONICAL_SURFACE ( 'NONE', #93559, 0.09999999999999982514, 0.003490658503988666988 ) ;
#97670=VERTEX_POINT ( 'NONE', #121106 ) ;
#97672=CARTESIAN_POINT ( 'NONE',  ( 3.349999999999941025, 2.500000000000000000, 7.088010851410848190 ) ) ;
#97673=CIRCLE ( 'NONE', #30796, 0.09999999999999982514 ) ;
#97674=DIRECTION ( 'NONE',  ( 0.000000000000000000, 0.000000000000000000, -1.000000000000000000 ) ) ;
#97675=CARTESIAN_POINT ( 'NONE',  ( 6.649999999999929301, 2.500000000000000000, 6.495190528383297135 ) ) ;
#97676=ORIENTED_EDGE ( 'NONE', *, *, #117370, .T. ) ;
#97677=AXIS2_PLACEMENT_3D ( 'NONE', #109547, #97786, #7457 ) ;
#97678=CARTESIAN_POINT ( 'NONE',  ( -1.650000000000035216, 2.500000000000000000, -1.472243186433550122 ) ) ;
#97679=FACE_OUTER_BOUND ( 'NONE', #74003, .T. ) ;
#97680=ORIENTED_EDGE ( 'NONE', *, *, #39930, .F. ) ;
#97681=CARTESIAN_POINT ( 'NONE',  ( -2.100000000000033396, 12.50000000000000000, -3.637306695894650055 ) ) ;
#97682=CARTESIAN_POINT ( 'NONE',  ( 3.549999999999944755, 2.500000000000000000, -2.511473670974877948 ) ) ;
#97683=DIRECTION ( 'NONE',  ( 0.000000000000000000, 1.000000000000000000, 0.000000000000000000 ) ) ;
#97685=FACE_OUTER_BOUND ( 'NONE', #48247, .T. ) ;
#97686=VERTEX_POINT ( 'NONE', #119820 ) ;
#97687=DIRECTION ( 'NONE',  ( 0.000000000000000000, 0.000000000000000000, 1.000000000000000000 ) ) ;
#97688=DIRECTION ( 'NONE',  ( -0.000000000000000000, -1.000000000000000000, -0.000000000000000000 ) ) ;
#97689=CIRCLE ( 'NONE', #35029, 0.06509327318403745899 ) ;
#97690=CARTESIAN_POINT ( 'NONE',  ( 3.949999999999939782, 12.50000000000000000, 2.511473670974873507 ) ) ;
#97691=ORIENTED_EDGE ( 'NONE', *, *, #97139, .F. ) ;
#97692=ADVANCED_FACE ( 'NONE', ( #110010 ), #3319, .T. ) ;
#97693=CARTESIAN_POINT ( 'NONE',  ( -9.550000000000002487, 2.500000000000000000, 6.495190528383297135 ) ) ;
#97694=VERTEX_POINT ( 'NONE', #20974 ) ;
#97695=EDGE_CURVE ( 'NONE', #18337, #72434, #118331, .T. ) ;
#97696=CARTESIAN_POINT ( 'NONE',  ( -11.24999999999996270, 2.500000000000000000, 2.165063509461097713 ) ) ;
#97697=EDGE_CURVE ( 'NONE', #11408, #24701, #61561, .T. ) ;
#97698=ORIENTED_EDGE ( 'NONE', *, *, #81965, .F. ) ;
#97699=DIRECTION ( 'NONE',  ( 0.000000000000000000, 1.000000000000000000, 0.000000000000000000 ) ) ;
#97700=AXIS2_PLACEMENT_3D ( 'NONE', #89882, #40151, #105167 ) ;
#97701=VECTOR ( 'NONE', #127938, 1000.000000000000000 ) ;
#97702=ORIENTED_EDGE ( 'NONE', *, *, #33345, .F. ) ;
#97703=FACE_OUTER_BOUND ( 'NONE', #21881, .T. ) ;
#97704=DIRECTION ( 'NONE',  ( 0.000000000000000000, 1.000000000000000000, 0.000000000000000000 ) ) ;
#97706=ADVANCED_FACE ( 'NONE', ( #89080 ), #47251, .T. ) ;
#97707=ORIENTED_EDGE ( 'NONE', *, *, #99936, .T. ) ;
#97708=VERTEX_POINT ( 'NONE', #39358 ) ;
#97709=EDGE_CURVE ( 'NONE', #108298, #8661, #21625, .T. ) ;
#97710=DIRECTION ( 'NONE',  ( 0.000000000000000000, 0.000000000000000000, 1.000000000000000000 ) ) ;
#97711=CARTESIAN_POINT ( 'NONE',  ( -11.64999999999999680, 2.500000000000000000, 5.702370205355745014 ) ) ;
#97712=ORIENTED_EDGE ( 'NONE', *, *, #73505, .T. ) ;
#97713=CONICAL_SURFACE ( 'NONE', #74742, 0.1000000000000002554, 0.003490658503988666988 ) ;
#97714=CONICAL_SURFACE ( 'NONE', #87237, 0.09999999999999982514, 0.003490658503988666988 ) ;
#97715=DIRECTION ( 'NONE',  ( -0.000000000000000000, 1.000000000000000000, -0.000000000000000000 ) ) ;
#97716=DIRECTION ( 'NONE',  ( 0.000000000000000000, 0.000000000000000000, 1.000000000000000000 ) ) ;
#97717=AXIS2_PLACEMENT_3D ( 'NONE', #101647, #23082, #11962 ) ;
#97719=DIRECTION ( 'NONE',  ( 0.000000000000000000, 0.000000000000000000, -1.000000000000000000 ) ) ;
#97720=DIRECTION ( 'NONE',  ( -4.274815082592931898E-19, -0.9999939076577903929, -0.003490651415223739937 ) ) ;
#97721=CARTESIAN_POINT ( 'NONE',  ( -6.450000000000019718, 2.500000000000000000, -6.248780366869526759 ) ) ;
#97722=CIRCLE ( 'NONE', #114176, 0.09999999999999982514 ) ;
#97723=AXIS2_PLACEMENT_3D ( 'NONE', #99680, #12558, #80684 ) ;
#97724=ORIENTED_EDGE ( 'NONE', *, *, #101984, .T. ) ;
#97725=ORIENTED_EDGE ( 'NONE', *, *, #38679, .T. ) ;
#97726=ORIENTED_EDGE ( 'NONE', *, *, #47535, .T. ) ;
#97727=EDGE_LOOP ( 'NONE', ( #125889, #9616, #53347, #99685 ) ) ;
#97728=CARTESIAN_POINT ( 'NONE',  ( -3.950000000000026379, 2.500000000000000000, 2.611473670974873151 ) ) ;
#97729=CARTESIAN_POINT ( 'NONE',  ( -11.44999999999999751, 2.500000000000000000, 2.511473670974873507 ) ) ;
#97730=CARTESIAN_POINT ( 'NONE',  ( 8.349999999999919709, 2.500000000000000000, 5.802370205355744659 ) ) ;
#97731=EDGE_LOOP ( 'NONE', ( #40684, #33648 ) ) ;
#97732=FACE_BOUND ( 'NONE', #97731, .T. ) ;
#97733=EDGE_LOOP ( 'NONE', ( #128116, #12778, #35747, #66785 ) ) ;
#97734=DIRECTION ( 'NONE',  ( -0.000000000000000000, -1.000000000000000000, -0.000000000000000000 ) ) ;
#97735=DIRECTION ( 'NONE',  ( 0.000000000000000000, 0.000000000000000000, 1.000000000000000000 ) ) ;
#97736=CARTESIAN_POINT ( 'NONE',  ( 3.949999999999942446, 2.500000000000000000, -2.411473670974877859 ) ) ;
#97737=VECTOR ( 'NONE', #93247, 1000.000000000000000 ) ;
#97738=DIRECTION ( 'NONE',  ( -0.000000000000000000, 1.000000000000000000, -0.000000000000000000 ) ) ;
#97739=CARTESIAN_POINT ( 'NONE',  ( 11.64999999999990798, 2.500000000000000000, 5.702370205355745014 ) ) ;
#97740=CIRCLE ( 'NONE', #106158, 0.06509327318403745899 ) ;
#97741=DIRECTION ( 'NONE',  ( 0.000000000000000000, 1.000000000000000000, 0.000000000000000000 ) ) ;
#97742=DIRECTION ( 'NONE',  ( 0.000000000000000000, -0.000000000000000000, 1.000000000000000000 ) ) ;
#97743=DIRECTION ( 'NONE',  ( 0.000000000000000000, 0.000000000000000000, 1.000000000000000000 ) ) ;
#97744=DIRECTION ( 'NONE',  ( -4.274815082592931898E-19, -0.9999939076577903929, -0.003490651415223739937 ) ) ;
#97745=AXIS2_PLACEMENT_3D ( 'NONE', #56210, #86968, #16902 ) ;
#97747=LINE ( 'NONE', #108211, #48089 ) ;
#97748=ORIENTED_EDGE ( 'NONE', *, *, #88684, .F. ) ;
#97749=CIRCLE ( 'NONE', #7856, 0.09999999999999982514 ) ;
#97750=ORIENTED_EDGE ( 'NONE', *, *, #82978, .T. ) ;
#97751=ORIENTED_EDGE ( 'NONE', *, *, #122754, .F. ) ;
#97752=ORIENTED_EDGE ( 'NONE', *, *, #119921, .T. ) ;
#97753=CARTESIAN_POINT ( 'NONE',  ( 10.84999999999991260, 2.500000000000000000, -1.472243186433550122 ) ) ;
#97754=ADVANCED_FACE ( 'NONE', ( #81194 ), #72383, .T. ) ;
#97755=PLANE ( 'NONE',  #6708 ) ;
#97756=EDGE_CURVE ( 'NONE', #127901, #56703, #19025, .T. ) ;
#97757=ORIENTED_EDGE ( 'NONE', *, *, #20443, .F. ) ;
#97758=VERTEX_POINT ( 'NONE', #98885 ) ;
#97759=VECTOR ( 'NONE', #75514, 1000.000000000000000 ) ;
#97760=ORIENTED_EDGE ( 'NONE', *, *, #43108, .T. ) ;
#97761=ADVANCED_FACE ( 'NONE', ( #31452 ), #9582, .T. ) ;
#97762=FACE_OUTER_BOUND ( 'NONE', #122414, .T. ) ;
#97763=VECTOR ( 'NONE', #82133, 1000.000000000000000 ) ;
#97764=AXIS2_PLACEMENT_3D ( 'NONE', #126832, #57448, #56142 ) ;
#97765=CARTESIAN_POINT ( 'NONE',  ( 14.54999999999989591, 12.50000000000000000, 2.230156782645134950 ) ) ;
#97766=DIRECTION ( 'NONE',  ( -0.000000000000000000, -1.000000000000000000, -0.000000000000000000 ) ) ;
#97767=EDGE_CURVE ( 'NONE', #127558, #62304, #40998, .T. ) ;
#97768=DIRECTION ( 'NONE',  ( 0.000000000000000000, 0.000000000000000000, -1.000000000000000000 ) ) ;
#97770=DIRECTION ( 'NONE',  ( -0.000000000000000000, 1.000000000000000000, -0.000000000000000000 ) ) ;
#97771=CARTESIAN_POINT ( 'NONE',  ( -13.74999999999998757, 2.500000000000000000, -2.857883832488651521 ) ) ;
#97772=AXIS2_PLACEMENT_3D ( 'NONE', #96006, #116274, #45631 ) ;
#97773=ORIENTED_EDGE ( 'NONE', *, *, #7981, .T. ) ;
#97774=CARTESIAN_POINT ( 'NONE',  ( 13.94999999999989804, 12.50000000000000000, 1.818653347947321475 ) ) ;
#97775=EDGE_CURVE ( 'NONE', #126779, #108066, #70225, .T. ) ;
#97776=ORIENTED_EDGE ( 'NONE', *, *, #76038, .F. ) ;
#97777=AXIS2_PLACEMENT_3D ( 'NONE', #2155, #100370, #30358 ) ;
#97778=EDGE_CURVE ( 'NONE', #100183, #123328, #63960, .T. ) ;
#97779=ORIENTED_EDGE ( 'NONE', *, *, #9483, .F. ) ;
#97780=EDGE_LOOP ( 'NONE', ( #108992, #117550 ) ) ;
#97781=CARTESIAN_POINT ( 'NONE',  ( -7.900000000000014566, 2.500000000000000000, -0.1000000000000022815 ) ) ;
#97782=ORIENTED_EDGE ( 'NONE', *, *, #28576, .T. ) ;
#97784=ADVANCED_FACE ( 'NONE', ( #63481 ), #83132, .T. ) ;
#97785=DIRECTION ( 'NONE',  ( 0.000000000000000000, 0.000000000000000000, 1.000000000000000000 ) ) ;
#97786=DIRECTION ( 'NONE',  ( -0.000000000000000000, -1.000000000000000000, -0.000000000000000000 ) ) ;
#97788=DIRECTION ( 'NONE',  ( 0.000000000000000000, 1.000000000000000000, 0.000000000000000000 ) ) ;
#97789=DIRECTION ( 'NONE',  ( 0.000000000000000000, 1.000000000000000000, 0.000000000000000000 ) ) ;
#97790=ORIENTED_EDGE ( 'NONE', *, *, #111446, .F. ) ;
#97791=CARTESIAN_POINT ( 'NONE',  ( -2.900000000000030109, 12.50000000000000000, -3.637306695894650055 ) ) ;
#97792=ORIENTED_EDGE ( 'NONE', *, *, #59937, .F. ) ;
#97793=DIRECTION ( 'NONE',  ( 0.000000000000000000, 0.000000000000000000, 1.000000000000000000 ) ) ;
#97794=VERTEX_POINT ( 'NONE', #3272 ) ;
#97796=CARTESIAN_POINT ( 'NONE',  ( -11.84999999999999609, 2.500000000000000000, 6.841600689897072485 ) ) ;
#97797=ORIENTED_EDGE ( 'NONE', *, *, #124061, .T. ) ;
#97798=LINE ( 'NONE', #8755, #121911 ) ;
#97799=DIRECTION ( 'NONE',  ( 0.000000000000000000, 0.000000000000000000, -1.000000000000000000 ) ) ;
#97800=ORIENTED_EDGE ( 'NONE', *, *, #95593, .T. ) ;
#97801=CIRCLE ( 'NONE', #18377, 0.06509327318403745899 ) ;
#97802=FACE_OUTER_BOUND ( 'NONE', #121264, .T. ) ;
#97803=ORIENTED_EDGE ( 'NONE', *, *, #6378, .T. ) ;
#97804=EDGE_LOOP ( 'NONE', ( #7542, #28899 ) ) ;
#97805=FACE_OUTER_BOUND ( 'NONE', #8357, .T. ) ;
#97806=DIRECTION ( 'NONE',  ( 0.000000000000000000, 1.000000000000000000, 0.000000000000000000 ) ) ;
#97808=CARTESIAN_POINT ( 'NONE',  ( 6.649999999999928413, 2.500000000000000000, 2.857883832488649301 ) ) ;
#97809=VECTOR ( 'NONE', #117397, 1000.000000000000000 ) ;
#97810=AXIS2_PLACEMENT_3D ( 'NONE', #11158, #120481, #111962 ) ;
#97811=LINE ( 'NONE', #76253, #10251 ) ;
#97812=EDGE_CURVE ( 'NONE', #2544, #18098, #111942, .T. ) ;
#97813=CIRCLE ( 'NONE', #112683, 0.06509327318403745899 ) ;
#97814=DIRECTION ( 'NONE',  ( 0.000000000000000000, 0.000000000000000000, -1.000000000000000000 ) ) ;
#97815=VERTEX_POINT ( 'NONE', #62209 ) ;
#97816=DIRECTION ( 'NONE',  ( -0.000000000000000000, -1.000000000000000000, -0.000000000000000000 ) ) ;
#97817=DIRECTION ( 'NONE',  ( 0.000000000000000000, 1.000000000000000000, 0.000000000000000000 ) ) ;
#97818=ORIENTED_EDGE ( 'NONE', *, *, #90020, .T. ) ;
#97819=AXIS2_PLACEMENT_3D ( 'NONE', #68347, #106967, #8762 ) ;
#97820=FACE_OUTER_BOUND ( 'NONE', #10684, .T. ) ;
#97821=DIRECTION ( 'NONE',  ( 0.000000000000000000, 0.000000000000000000, 1.000000000000000000 ) ) ;
#97822=DIRECTION ( 'NONE',  ( 0.000000000000000000, 1.000000000000000000, 0.000000000000000000 ) ) ;
#97823=CARTESIAN_POINT ( 'NONE',  ( 9.349999999999916156, 12.50000000000000000, 6.841600689897072485 ) ) ;
#97824=DIRECTION ( 'NONE',  ( 0.000000000000000000, -0.9999939076577903929, 0.003490651415223739937 ) ) ;
#97825=EDGE_LOOP ( 'NONE', ( #58919, #23371 ) ) ;
#97826=AXIS2_PLACEMENT_3D ( 'NONE', #41375, #81285, #89166 ) ;
#97827=DIRECTION ( 'NONE',  ( 0.000000000000000000, 0.000000000000000000, -1.000000000000000000 ) ) ;
#97828=DIRECTION ( 'NONE',  ( 0.000000000000000000, 0.000000000000000000, 1.000000000000000000 ) ) ;
#97829=AXIS2_PLACEMENT_3D ( 'NONE', #68299, #15967, #108231 ) ;
#97830=ORIENTED_EDGE ( 'NONE', *, *, #80290, .T. ) ;
#97831=CONICAL_SURFACE ( 'NONE', #114555, 0.1000000000000002554, 0.003490658503988666988 ) ;
#97832=DIRECTION ( 'NONE',  ( 0.000000000000000000, 0.000000000000000000, -1.000000000000000000 ) ) ;
#97833=CIRCLE ( 'NONE', #112436, 0.09999999999999982514 ) ;
#97834=EDGE_LOOP ( 'NONE', ( #48739, #52825 ) ) ;
#97835=ORIENTED_EDGE ( 'NONE', *, *, #58832, .T. ) ;
#97836=DIRECTION ( 'NONE',  ( 0.000000000000000000, -0.9999939076577903929, 0.003490651415223739937 ) ) ;
#97837=CIRCLE ( 'NONE', #128989, 0.06509327318403745899 ) ;
#97838=ORIENTED_EDGE ( 'NONE', *, *, #111637, .F. ) ;
#97840=DIRECTION ( 'NONE',  ( 0.000000000000000000, 0.000000000000000000, 1.000000000000000000 ) ) ;
#97841=DIRECTION ( 'NONE',  ( 0.000000000000000000, 0.000000000000000000, 1.000000000000000000 ) ) ;
#97842=ORIENTED_EDGE ( 'NONE', *, *, #120970, .F. ) ;
#97843=EDGE_CURVE ( 'NONE', #56218, #42111, #120399, .T. ) ;
#97844=DIRECTION ( 'NONE',  ( 0.000000000000000000, -0.000000000000000000, 1.000000000000000000 ) ) ;
#97845=LINE ( 'NONE', #119411, #84948 ) ;
#97846=VERTEX_POINT ( 'NONE', #93585 ) ;
#97847=DIRECTION ( 'NONE',  ( 0.000000000000000000, 0.000000000000000000, 1.000000000000000000 ) ) ;
#97848=CIRCLE ( 'NONE', #30994, 0.06509327318403745899 ) ;
#97849=EDGE_CURVE ( 'NONE', #31054, #106287, #2605, .T. ) ;
#97850=DIRECTION ( 'NONE',  ( 0.000000000000000000, -0.000000000000000000, 1.000000000000000000 ) ) ;
#97851=EDGE_CURVE ( 'NONE', #119823, #14270, #101478, .T. ) ;
#97852=ORIENTED_EDGE ( 'NONE', *, *, #64069, .F. ) ;
#97853=VECTOR ( 'NONE', #118612, 1000.000000000000000 ) ;
#97854=VERTEX_POINT ( 'NONE', #122411 ) ;
#97855=VERTEX_POINT ( 'NONE', #64117 ) ;
#97856=CARTESIAN_POINT ( 'NONE',  ( -8.550000000000011369, 12.50000000000000000, 1.818653347947321475 ) ) ;
#97857=CARTESIAN_POINT ( 'NONE',  ( -1.650000000000034772, 2.500000000000000000, 2.165063509461097713 ) ) ;
#97858=EDGE_CURVE ( 'NONE', #50747, #112355, #54299, .T. ) ;
#97859=EDGE_CURVE ( 'NONE', #121535, #89650, #32753, .T. ) ;
#97860=DIRECTION ( 'NONE',  ( 0.000000000000000000, 0.000000000000000000, 1.000000000000000000 ) ) ;
#97861=ADVANCED_FACE ( 'NONE', ( #22919 ), #7511, .T. ) ;
#97862=FACE_BOUND ( 'NONE', #108970, .T. ) ;
#97863=ORIENTED_EDGE ( 'NONE', *, *, #9581, .T. ) ;
#97864=EDGE_CURVE ( 'NONE', #127371, #96017, #99476, .T. ) ;
#97865=EDGE_CURVE ( 'NONE', #92342, #58017, #78650, .T. ) ;
#97866=LINE ( 'NONE', #27835, #84631 ) ;
#97867=CARTESIAN_POINT ( 'NONE',  ( -7.100000000000017408, 2.500000000000000000, -3.637306695894650055 ) ) ;
#97869=LINE ( 'NONE', #56636, #34564 ) ;
#97870=DIRECTION ( 'NONE',  ( 0.000000000000000000, 0.000000000000000000, 1.000000000000000000 ) ) ;
#97871=FACE_OUTER_BOUND ( 'NONE', #106118, .T. ) ;
#97872=ADVANCED_FACE ( 'NONE', ( #66048 ), #97400, .T. ) ;
#97873=LINE ( 'NONE', #128665, #82651 ) ;
#97874=CARTESIAN_POINT ( 'NONE',  ( -5.850000000000021849, 2.500000000000000000, -7.188010851410854052 ) ) ;
#97875=CIRCLE ( 'NONE', #110496, 0.09999999999999982514 ) ;
#97876=EDGE_LOOP ( 'NONE', ( #96791, #93475 ) ) ;
#97878=ORIENTED_EDGE ( 'NONE', *, *, #104431, .T. ) ;
#97879=AXIS2_PLACEMENT_3D ( 'NONE', #1316, #110631, #60275 ) ;
#97880=AXIS2_PLACEMENT_3D ( 'NONE', #44483, #104054, #14363 ) ;
#97881=ORIENTED_EDGE ( 'NONE', *, *, #123403, .F. ) ;
#97882=VERTEX_POINT ( 'NONE', #126918 ) ;
#97883=DIRECTION ( 'NONE',  ( 0.000000000000000000, 0.000000000000000000, 1.000000000000000000 ) ) ;
#97884=DIRECTION ( 'NONE',  ( -0.000000000000000000, 1.000000000000000000, -0.000000000000000000 ) ) ;
#97885=ORIENTED_EDGE ( 'NONE', *, *, #41521, .F. ) ;
#97886=FACE_BOUND ( 'NONE', #86894, .T. ) ;
#97887=CARTESIAN_POINT ( 'NONE',  ( -11.25000000000000000, 12.50000000000000000, -2.857883832488649745 ) ) ;
#97888=CIRCLE ( 'NONE', #116757, 0.06509327318403745899 ) ;
#97889=DIRECTION ( 'NONE',  ( 0.000000000000000000, -0.000000000000000000, 1.000000000000000000 ) ) ;
#97891=DIRECTION ( 'NONE',  ( 0.000000000000000000, 1.000000000000000000, 0.000000000000000000 ) ) ;
#97892=DIRECTION ( 'NONE',  ( 0.000000000000000000, -0.000000000000000000, 1.000000000000000000 ) ) ;
#97893=VERTEX_POINT ( 'NONE', #107264 ) ;
#97894=CARTESIAN_POINT ( 'NONE',  ( 8.949999999999921130, 2.500000000000000000, -6.841600689897078702 ) ) ;
#97895=AXIS2_PLACEMENT_3D ( 'NONE', #98650, #49586, #128801 ) ;
#97896=ORIENTED_EDGE ( 'NONE', *, *, #54766, .F. ) ;
#97897=AXIS2_PLACEMENT_3D ( 'NONE', #39293, #119740, #87699 ) ;
#97898=ORIENTED_EDGE ( 'NONE', *, *, #17313, .T. ) ;
#97899=VERTEX_POINT ( 'NONE', #94870 ) ;
#97900=PLANE ( 'NONE',  #48472 ) ;
#97901=PLANE ( 'NONE',  #56803 ) ;
#97902=DIRECTION ( 'NONE',  ( 0.000000000000000000, -0.9999939076577903929, 0.003490651415223739937 ) ) ;
#97904=ORIENTED_EDGE ( 'NONE', *, *, #2588, .T. ) ;
#97905=CARTESIAN_POINT ( 'NONE',  ( -9.350000000000008527, 2.500000000000000000, -6.048780366869521252 ) ) ;
#97906=EDGE_CURVE ( 'NONE', #50060, #67824, #87617, .T. ) ;
#97907=AXIS2_PLACEMENT_3D ( 'NONE', #103383, #72641, #115101 ) ;
#97908=CARTESIAN_POINT ( 'NONE',  ( -1.450000000000035039, 12.50000000000000000, -6.776507416713039689 ) ) ;
#97909=EDGE_CURVE ( 'NONE', #21143, #87403, #20058, .T. ) ;
#97910=CARTESIAN_POINT ( 'NONE',  ( 7.049999999999930544, 2.500000000000000000, -6.595190528383302109 ) ) ;
#97912=DIRECTION ( 'NONE',  ( 0.000000000000000000, 0.000000000000000000, 1.000000000000000000 ) ) ;
#97913=LINE ( 'NONE', #109012, #25847 ) ;
#97914=AXIS2_PLACEMENT_3D ( 'NONE', #104258, #125809, #105551 ) ;
#97915=DIRECTION ( 'NONE',  ( 0.000000000000000000, 1.000000000000000000, 0.000000000000000000 ) ) ;
#97916=ADVANCED_FACE ( 'NONE', ( #76527 ), #11721, .T. ) ;
#97917=VERTEX_POINT ( 'NONE', #116430 ) ;
#97918=DIRECTION ( 'NONE',  ( 0.000000000000000000, 0.000000000000000000, -1.000000000000000000 ) ) ;
#97919=EDGE_CURVE ( 'NONE', #115380, #41348, #28464, .T. ) ;
#97920=AXIS2_PLACEMENT_3D ( 'NONE', #96826, #78512, #58226 ) ;
#97921=EDGE_CURVE ( 'NONE', #95937, #118189, #55642, .T. ) ;
#97922=ORIENTED_EDGE ( 'NONE', *, *, #38676, .T. ) ;
#97923=EDGE_CURVE ( 'NONE', #94609, #24381, #125785, .T. ) ;
#97924=EDGE_LOOP ( 'NONE', ( #74900, #106861 ) ) ;
#97926=DIRECTION ( 'NONE',  ( -0.000000000000000000, -1.000000000000000000, -0.000000000000000000 ) ) ;
#97927=DIRECTION ( 'NONE',  ( 0.000000000000000000, 1.000000000000000000, 0.000000000000000000 ) ) ;
#97928=DIRECTION ( 'NONE',  ( 0.000000000000000000, 1.000000000000000000, 0.000000000000000000 ) ) ;
#97929=VERTEX_POINT ( 'NONE', #14987 ) ;
#97930=CIRCLE ( 'NONE', #81306, 0.06509327318403741736 ) ;
#97931=ADVANCED_FACE ( 'NONE', ( #96786 ), #53502, .T. ) ;
#97932=VERTEX_POINT ( 'NONE', #75863 ) ;
#97934=AXIS2_PLACEMENT_3D ( 'NONE', #17824, #47948, #87847 ) ;
#97935=DIRECTION ( 'NONE',  ( 0.000000000000000000, 0.000000000000000000, 1.000000000000000000 ) ) ;
#97936=CARTESIAN_POINT ( 'NONE',  ( -14.34999999999998543, 2.500000000000000000, 1.918653347947325338 ) ) ;
#97937=ORIENTED_EDGE ( 'NONE', *, *, #62451, .T. ) ;
#97938=ORIENTED_EDGE ( 'NONE', *, *, #79808, .T. ) ;
#97939=CARTESIAN_POINT ( 'NONE',  ( 7.049999999999928768, 12.50000000000000000, -2.165063509461101710 ) ) ;
#97940=VECTOR ( 'NONE', #89208, 1000.000000000000000 ) ;
#97941=ORIENTED_EDGE ( 'NONE', *, *, #78020, .F. ) ;
#97942=CARTESIAN_POINT ( 'NONE',  ( -4.350000000000023626, 2.500000000000000000, -1.918653347947325782 ) ) ;
#97943=CARTESIAN_POINT ( 'NONE',  ( -7.700000000000010836, 2.500000000000000000, 3.883716857408421319 ) ) ;
#97944=ORIENTED_EDGE ( 'NONE', *, *, #107795, .T. ) ;
#97945=DIRECTION ( 'NONE',  ( 0.000000000000000000, 0.000000000000000000, 1.000000000000000000 ) ) ;
#97946=FACE_OUTER_BOUND ( 'NONE', #59670, .T. ) ;
#97947=CARTESIAN_POINT ( 'NONE',  ( 13.34999999999989662, 2.500000000000000000, -1.472243186433550122 ) ) ;
#97948=AXIS2_PLACEMENT_3D ( 'NONE', #12864, #54105, #45582 ) ;
#97949=EDGE_CURVE ( 'NONE', #110675, #70171, #109938, .T. ) ;
#97950=CARTESIAN_POINT ( 'NONE',  ( -14.19999999999998685, 2.500000000000000000, -1.084202172485504434E-16 ) ) ;
#97951=ORIENTED_EDGE ( 'NONE', *, *, #60956, .T. ) ;
#97952=DIRECTION ( 'NONE',  ( 0.000000000000000000, 0.000000000000000000, -1.000000000000000000 ) ) ;
#97953=VECTOR ( 'NONE', #65027, 1000.000000000000000 ) ;
#97954=AXIS2_PLACEMENT_3D ( 'NONE', #116979, #105895, #107166 ) ;
#97955=VERTEX_POINT ( 'NONE', #97443 ) ;
#97956=EDGE_LOOP ( 'NONE', ( #97420, #42707 ) ) ;
#97957=CARTESIAN_POINT ( 'NONE',  ( 5.599999999999933031, 12.50000000000000000, 0.2813168883297361700 ) ) ;
#97958=DIRECTION ( 'NONE',  ( 0.000000000000000000, 1.000000000000000000, 0.000000000000000000 ) ) ;
#97959=DIRECTION ( 'NONE',  ( -4.274815082592931898E-19, -0.9999939076577903929, -0.003490651415223739937 ) ) ;
#97960=CARTESIAN_POINT ( 'NONE',  ( 11.44999999999990514, 2.500000000000000000, 2.511473670974873507 ) ) ;
#97961=CARTESIAN_POINT ( 'NONE',  ( -11.05000000000000071, 2.500000000000000000, 2.511473670974873507 ) ) ;
#97962=CARTESIAN_POINT ( 'NONE',  ( -12.09999999999999609, 12.50000000000000000, -0.6928203230275501445 ) ) ;
#97963=DIRECTION ( 'NONE',  ( 0.000000000000000000, 0.000000000000000000, 1.000000000000000000 ) ) ;
#97964=ADVANCED_FACE ( 'NONE', ( #77790 ), #115794, .T. ) ;
#97965=DIRECTION ( 'NONE',  ( 0.000000000000000000, 0.000000000000000000, 1.000000000000000000 ) ) ;
#97966=CARTESIAN_POINT ( 'NONE',  ( 9.149999999999915090, 2.500000000000000000, 6.595190528383296780 ) ) ;
#97967=AXIS2_PLACEMENT_3D ( 'NONE', #61675, #110747, #21080 ) ;
#97968=DIRECTION ( 'NONE',  ( -0.000000000000000000, -1.000000000000000000, -0.000000000000000000 ) ) ;
#97969=CIRCLE ( 'NONE', #14425, 0.06509327318403741736 ) ;
#97970=CIRCLE ( 'NONE', #68725, 0.06509327318403745899 ) ;
#97971=VERTEX_POINT ( 'NONE', #117706 ) ;
#97972=VECTOR ( 'NONE', #36469, 1000.000000000000000 ) ;
#97973=CARTESIAN_POINT ( 'NONE',  ( 10.64999999999991331, 12.50000000000000000, -1.818653347947325916 ) ) ;
#97974=EDGE_CURVE ( 'NONE', #36786, #52806, #54936, .T. ) ;
#97975=FACE_OUTER_BOUND ( 'NONE', #62873, .T. ) ;
#97976=CARTESIAN_POINT ( 'NONE',  ( 9.349999999999916156, 2.500000000000000000, 6.148780366869520009 ) ) ;
#97977=FACE_OUTER_BOUND ( 'NONE', #36891, .T. ) ;
#97978=DIRECTION ( 'NONE',  ( 0.000000000000000000, 0.000000000000000000, -1.000000000000000000 ) ) ;
#97979=AXIS2_PLACEMENT_3D ( 'NONE', #36768, #28227, #16441 ) ;
#97980=ORIENTED_EDGE ( 'NONE', *, *, #98186, .T. ) ;
#97981=AXIS2_PLACEMENT_3D ( 'NONE', #61430, #82358, #119673 ) ;
#97982=CARTESIAN_POINT ( 'NONE',  ( 7.099999999999928590, 2.500000000000000000, 3.737306695894644371 ) ) ;
#97983=FACE_OUTER_BOUND ( 'NONE', #39769, .T. ) ;
#97984=DIRECTION ( 'NONE',  ( 0.000000000000000000, 0.000000000000000000, 1.000000000000000000 ) ) ;
#97985=ORIENTED_EDGE ( 'NONE', *, *, #113262, .T. ) ;
#97986=VECTOR ( 'NONE', #74361, 1000.000000000000000 ) ;
#97987=ORIENTED_EDGE ( 'NONE', *, *, #60039, .F. ) ;
#97988=PLANE ( 'NONE',  #115715 ) ;
#97989=VERTEX_POINT ( 'NONE', #26139 ) ;
#97990=ORIENTED_EDGE ( 'NONE', *, *, #24128, .T. ) ;
#97991=EDGE_LOOP ( 'NONE', ( #30365, #63378, #109863, #71200 ) ) ;
#97992=FACE_OUTER_BOUND ( 'NONE', #75672, .T. ) ;
#97993=CARTESIAN_POINT ( 'NONE',  ( 3.549999999999942091, 2.500000000000000000, 2.511473670974873507 ) ) ;
#97994=CARTESIAN_POINT ( 'NONE',  ( -4.800000000000024691, 2.500000000000000000, 4.676537180435972552 ) ) ;
#97995=DIRECTION ( 'NONE',  ( -4.274815082592931898E-19, -0.9999939076577903929, -0.003490651415223739937 ) ) ;
#97996=AXIS2_PLACEMENT_3D ( 'NONE', #11618, #69904, #19502 ) ;
#97997=EDGE_LOOP ( 'NONE', ( #40525, #125671 ) ) ;
#97998=ADVANCED_FACE ( 'NONE', ( #9062 ), #59493, .T. ) ;
#97999=DIRECTION ( 'NONE',  ( 0.000000000000000000, 1.000000000000000000, 0.000000000000000000 ) ) ;
#98000=ORIENTED_EDGE ( 'NONE', *, *, #34177, .F. ) ;
#98001=AXIS2_PLACEMENT_3D ( 'NONE', #87817, #117263, #97653 ) ;
#98002=DIRECTION ( 'NONE',  ( 0.000000000000000000, -0.000000000000000000, 1.000000000000000000 ) ) ;
#98003=CARTESIAN_POINT ( 'NONE',  ( 16.31260002278194321, -1.499999999999773515, -6.357732714000996488 ) ) ;
#98004=CARTESIAN_POINT ( 'NONE',  ( 19.40342015654644925, 2.551666867760719715, 4.359384978533469734 ) ) ;
#98005=CARTESIAN_POINT ( 'NONE',  ( -2.900000000000029665, 12.50000000000000000, 3.702399969078682407 ) ) ;
#98006=CARTESIAN_POINT ( 'NONE',  ( -3.749999999999991118, 2.500000000000000000, -2.165063509461101710 ) ) ;
#98007=ORIENTED_EDGE ( 'NONE', *, *, #82930, .T. ) ;
#98008=ORIENTED_EDGE ( 'NONE', *, *, #20431, .T. ) ;
#98009=ORIENTED_EDGE ( 'NONE', *, *, #56452, .T. ) ;
#98010=ORIENTED_EDGE ( 'NONE', *, *, #121149, .F. ) ;
#98011=ORIENTED_EDGE ( 'NONE', *, *, #26245, .T. ) ;
#98012=DIRECTION ( 'NONE',  ( 0.000000000000000000, -0.000000000000000000, 1.000000000000000000 ) ) ;
#98013=DIRECTION ( 'NONE',  ( 0.000000000000000000, 1.000000000000000000, 0.000000000000000000 ) ) ;
#98014=ADVANCED_FACE ( 'NONE', ( #29368 ), #18878, .T. ) ;
#98015=EDGE_CURVE ( 'NONE', #84709, #94668, #74516, .T. ) ;
#98016=CARTESIAN_POINT ( 'NONE',  ( -2.500000000000031086, 2.500000000000000000, 3.537306695894645081 ) ) ;
#98017=EDGE_CURVE ( 'NONE', #99630, #80752, #58188, .T. ) ;
#98018=FACE_BOUND ( 'NONE', #98782, .T. ) ;
#98019=EDGE_CURVE ( 'NONE', #60331, #96594, #93297, .T. ) ;
#98020=DIRECTION ( 'NONE',  ( 0.000000000000000000, 0.000000000000000000, 1.000000000000000000 ) ) ;
#98022=AXIS2_PLACEMENT_3D ( 'NONE', #105010, #64452, #122101 ) ;
#98023=CARTESIAN_POINT ( 'NONE',  ( -1.450000000000035039, 2.500000000000000000, -6.841600689897077814 ) ) ;
#98024=DIRECTION ( 'NONE',  ( 0.000000000000000000, -0.000000000000000000, 1.000000000000000000 ) ) ;
#98025=VECTOR ( 'NONE', #89000, 1000.000000000000000 ) ;
#98026=EDGE_CURVE ( 'NONE', #20666, #98359, #18067, .T. ) ;
#98028=CARTESIAN_POINT ( 'NONE',  ( 10.19999999999991225, 12.50000000000000000, 3.918623584224382839 ) ) ;
#98029=AXIS2_PLACEMENT_3D ( 'NONE', #52055, #69748, #20016 ) ;
#98031=CARTESIAN_POINT ( 'NONE',  ( 14.39999999999989555, 12.50000000000000000, 0.2813168883297362810 ) ) ;
#98032=EDGE_CURVE ( 'NONE', #52139, #88048, #88247, .T. ) ;
#98033=EDGE_CURVE ( 'NONE', #128319, #37369, #79114, .T. ) ;
#98034=PLANE ( 'NONE',  #107906 ) ;
#98035=CIRCLE ( 'NONE', #22850, 0.06509327318403745899 ) ;
#98036=ORIENTED_EDGE ( 'NONE', *, *, #67891, .F. ) ;
#98037=EDGE_LOOP ( 'NONE', ( #82643, #73272, #17648, #96685 ) ) ;
#98038=EDGE_LOOP ( 'NONE', ( #92878, #117366 ) ) ;
#98039=ORIENTED_EDGE ( 'NONE', *, *, #100556, .T. ) ;
#98040=VECTOR ( 'NONE', #40273, 1000.000000000000000 ) ;
#98042=CARTESIAN_POINT ( 'NONE',  ( -6.850000000000017408, 2.500000000000000000, -2.411473670974877859 ) ) ;
#98043=FACE_BOUND ( 'NONE', #19598, .T. ) ;
#98044=EDGE_CURVE ( 'NONE', #27644, #127171, #9669, .T. ) ;
#98045=DIRECTION ( 'NONE',  ( 0.000000000000000000, 1.000000000000000000, 0.000000000000000000 ) ) ;
#98046=AXIS2_PLACEMENT_3D ( 'NONE', #67068, #115536, #97841 ) ;
#98048=CARTESIAN_POINT ( 'NONE',  ( -9.350000000000008527, 12.50000000000000000, -6.213873640053559022 ) ) ;
#98049=DIRECTION ( 'NONE',  ( 0.000000000000000000, 0.000000000000000000, 1.000000000000000000 ) ) ;
#98050=DIRECTION ( 'NONE',  ( 0.000000000000000000, 0.000000000000000000, -1.000000000000000000 ) ) ;
#98051=VERTEX_POINT ( 'NONE', #108560 ) ;
#98053=CARTESIAN_POINT ( 'NONE',  ( -0.6000000000000388356, 12.50000000000000000, 4.676537180435972552 ) ) ;
#98054=ORIENTED_EDGE ( 'NONE', *, *, #99508, .T. ) ;
#98055=ORIENTED_EDGE ( 'NONE', *, *, #53322, .T. ) ;
#98057=DIRECTION ( 'NONE',  ( 0.000000000000000000, -0.000000000000000000, 1.000000000000000000 ) ) ;
#98058=PLANE ( 'NONE',  #89481 ) ;
#98059=CIRCLE ( 'NONE', #93960, 0.1000000000000002554 ) ;
#98060=DIRECTION ( 'NONE',  ( 0.000000000000000000, 1.000000000000000000, 0.000000000000000000 ) ) ;
#98061=AXIS2_PLACEMENT_3D ( 'NONE', #85719, #15024, #104087 ) ;
#98062=DIRECTION ( 'NONE',  ( 0.000000000000000000, 0.000000000000000000, 1.000000000000000000 ) ) ;
#98063=DIRECTION ( 'NONE',  ( 0.000000000000000000, 1.000000000000000000, 0.000000000000000000 ) ) ;
#98064=ORIENTED_EDGE ( 'NONE', *, *, #4214, .F. ) ;
#98065=ORIENTED_EDGE ( 'NONE', *, *, #128317, .F. ) ;
#98066=FACE_OUTER_BOUND ( 'NONE', #30629, .T. ) ;
#98067=CIRCLE ( 'NONE', #102201, 0.06509327318403745899 ) ;
#98068=EDGE_LOOP ( 'NONE', ( #102007, #68167, #74075, #33827 ) ) ;
#98069=CARTESIAN_POINT ( 'NONE',  ( 3.149999999999946176, 12.50000000000000000, -6.906693963081115051 ) ) ;
#98070=FACE_BOUND ( 'NONE', #92098, .T. ) ;
#98071=CONICAL_SURFACE ( 'NONE', #70979, 0.1000000000000002554, 0.003490658503988666988 ) ;
#98072=ADVANCED_FACE ( 'NONE', ( #10976 ), #30619, .T. ) ;
#98073=AXIS2_PLACEMENT_3D ( 'NONE', #111950, #13067, #73948 ) ;
#98074=ORIENTED_EDGE ( 'NONE', *, *, #102292, .F. ) ;
#98076=EDGE_CURVE ( 'NONE', #102847, #79650, #120487, .T. ) ;
#98077=VERTEX_POINT ( 'NONE', #38557 ) ;
#98078=FACE_OUTER_BOUND ( 'NONE', #7678, .T. ) ;
#98079=DIRECTION ( 'NONE',  ( -0.000000000000000000, 1.000000000000000000, -0.000000000000000000 ) ) ;
#98080=LINE ( 'NONE', #8401, #115575 ) ;
#98081=LINE ( 'NONE', #86316, #41210 ) ;
#98082=CIRCLE ( 'NONE', #102306, 0.1000000000000002554 ) ;
#98083=ORIENTED_EDGE ( 'NONE', *, *, #129182, .F. ) ;
#98084=EDGE_CURVE ( 'NONE', #77768, #53425, #26407, .T. ) ;
#98085=EDGE_LOOP ( 'NONE', ( #32477, #122797, #11436, #82319 ) ) ;
#98086=AXIS2_PLACEMENT_3D ( 'NONE', #22822, #62741, #20872 ) ;
#98087=ORIENTED_EDGE ( 'NONE', *, *, #87826, .T. ) ;
#98088=CARTESIAN_POINT ( 'NONE',  ( 2.099999999999947686, 2.500000000000000000, 5.022947341949748790 ) ) ;
#98090=CARTESIAN_POINT ( 'NONE',  ( 1.449999999999952660, 2.500000000000000000, -6.941600689897078347 ) ) ;
#98091=ORIENTED_EDGE ( 'NONE', *, *, #22743, .F. ) ;
#98092=VERTEX_POINT ( 'NONE', #49659 ) ;
#98093=ORIENTED_EDGE ( 'NONE', *, *, #82251, .F. ) ;
#98094=DIRECTION ( 'NONE',  ( -0.000000000000000000, -1.000000000000000000, -0.000000000000000000 ) ) ;
#98095=DIRECTION ( 'NONE',  ( 0.000000000000000000, 0.000000000000000000, 1.000000000000000000 ) ) ;
#98097=DIRECTION ( 'NONE',  ( 0.000000000000000000, 1.000000000000000000, 0.000000000000000000 ) ) ;
#98098=CARTESIAN_POINT ( 'NONE',  ( -0.8500000000000390576, 12.50000000000000000, -6.430097255199264339 ) ) ;
#98099=CARTESIAN_POINT ( 'NONE',  ( -6.650000000000014566, 2.500000000000000000, 5.802370205355744659 ) ) ;
#98100=DIRECTION ( 'NONE',  ( 0.000000000000000000, -0.9999939076577903929, 0.003490651415223739937 ) ) ;
#98101=AXIS2_PLACEMENT_3D ( 'NONE', #105658, #97117, #8084 ) ;
#98103=DIRECTION ( 'NONE',  ( -0.000000000000000000, 1.000000000000000000, -0.000000000000000000 ) ) ;
#98104=ORIENTED_EDGE ( 'NONE', *, *, #58155, .F. ) ;
#98105=ORIENTED_EDGE ( 'NONE', *, *, #91998, .T. ) ;
#98106=DIRECTION ( 'NONE',  ( 0.000000000000000000, -0.000000000000000000, 1.000000000000000000 ) ) ;
#98107=CARTESIAN_POINT ( 'NONE',  ( 0.8499999999999545697, 2.500000000000000000, -1.472243186433550122 ) ) ;
#98108=VERTEX_POINT ( 'NONE', #89560 ) ;
#98109=ORIENTED_EDGE ( 'NONE', *, *, #54703, .F. ) ;
#98111=CARTESIAN_POINT ( 'NONE',  ( 7.699999999999923794, 2.500000000000000000, -3.983716857408426293 ) ) ;
#98112=CIRCLE ( 'NONE', #14468, 0.06509327318403745899 ) ;
#98113=CARTESIAN_POINT ( 'NONE',  ( 2.500000000000001332, 2.392226903609813160, -9.521986658763280431 ) ) ;
#98114=DIRECTION ( 'NONE',  ( -0.000000000000000000, -1.000000000000000000, -0.000000000000000000 ) ) ;
#98115=DIRECTION ( 'NONE',  ( 0.000000000000000000, 0.000000000000000000, -1.000000000000000000 ) ) ;
#98116=CARTESIAN_POINT ( 'NONE',  ( -3.100000000000028511, 2.500000000000000000, 0.3464101615137736845 ) ) ;
#98117=ORIENTED_EDGE ( 'NONE', *, *, #114119, .F. ) ;
#98118=DIRECTION ( 'NONE',  ( 0.000000000000000000, 1.000000000000000000, 0.000000000000000000 ) ) ;
#98119=CIRCLE ( 'NONE', #119062, 0.06509327318403745899 ) ;
#98120=DIRECTION ( 'NONE',  ( 0.000000000000000000, 1.000000000000000000, 0.000000000000000000 ) ) ;
#98121=ORIENTED_EDGE ( 'NONE', *, *, #36990, .T. ) ;
#98122=AXIS2_PLACEMENT_3D ( 'NONE', #58708, #76420, #9603 ) ;
#98123=AXIS2_PLACEMENT_3D ( 'NONE', #36553, #58755, #7701 ) ;
#98124=ORIENTED_EDGE ( 'NONE', *, *, #50326, .T. ) ;
#98125=EDGE_CURVE ( 'NONE', #49878, #1609, #64050, .T. ) ;
#98126=AXIS2_PLACEMENT_3D ( 'NONE', #103041, #93240, #76818 ) ;
#98127=ORIENTED_EDGE ( 'NONE', *, *, #112479, .T. ) ;
#98129=EDGE_LOOP ( 'NONE', ( #108662, #111727 ) ) ;
#98130=LINE ( 'NONE', #96836, #39952 ) ;
#98131=DIRECTION ( 'NONE',  ( 0.000000000000000000, -0.9999939076577903929, 0.003490651415223739937 ) ) ;
#98132=CONICAL_SURFACE ( 'NONE', #102358, 0.09999999999999999167, 0.003490658503988666988 ) ;
#98133=ORIENTED_EDGE ( 'NONE', *, *, #32919, .T. ) ;
#98134=FACE_OUTER_BOUND ( 'NONE', #16768, .T. ) ;
#98135=DIRECTION ( 'NONE',  ( 0.000000000000000000, 0.000000000000000000, -1.000000000000000000 ) ) ;
#98136=CARTESIAN_POINT ( 'NONE',  ( -6.505213034913026604E-15, 12.50000000000000000, 4.330127018922196314 ) ) ;
#98138=EDGE_LOOP ( 'NONE', ( #14560, #12479, #113685, #42062 ) ) ;
#98139=EDGE_CURVE ( 'NONE', #80664, #33748, #90182, .T. ) ;
#98140=DIRECTION ( 'NONE',  ( -4.274815082592931898E-19, -0.9999939076577903929, -0.003490651415223739937 ) ) ;
#98141=CARTESIAN_POINT ( 'NONE',  ( 0.5999999999999560130, 12.50000000000000000, -3.983716857408426293 ) ) ;
#98142=VERTEX_POINT ( 'NONE', #58818 ) ;
#98143=VERTEX_POINT ( 'NONE', #520 ) ;
#98144=EDGE_LOOP ( 'NONE', ( #58602, #76497 ) ) ;
#98145=AXIS2_PLACEMENT_3D ( 'NONE', #106903, #7409, #28366 ) ;
#98146=FACE_OUTER_BOUND ( 'NONE', #117151, .T. ) ;
#98147=DIRECTION ( 'NONE',  ( 0.000000000000000000, -0.9999939076577903929, 0.003490651415223739937 ) ) ;
#98148=AXIS2_PLACEMENT_3D ( 'NONE', #12658, #4127, #52596 ) ;
#98149=AXIS2_PLACEMENT_3D ( 'NONE', #58699, #26664, #98595 ) ;
#98150=EDGE_CURVE ( 'NONE', #116591, #38872, #89098, .T. ) ;
#98151=ORIENTED_EDGE ( 'NONE', *, *, #65545, .F. ) ;
#98152=CARTESIAN_POINT ( 'NONE',  ( -1.650000000000035216, 2.500000000000000000, -1.372243186433550033 ) ) ;
#98153=CARTESIAN_POINT ( 'NONE',  ( -9.200000000000006395, 2.500000000000000000, 4.430127018922196847 ) ) ;
#98154=DIRECTION ( 'NONE',  ( 0.000000000000000000, -0.9999939076577903929, 0.003490651415223739937 ) ) ;
#98155=DIRECTION ( 'NONE',  ( -0.000000000000000000, 1.000000000000000000, -0.000000000000000000 ) ) ;
#98156=AXIS2_PLACEMENT_3D ( 'NONE', #49516, #89425, #119519 ) ;
#98157=CONICAL_SURFACE ( 'NONE', #114884, 0.1000000000000002554, 0.003490658503988666988 ) ;
#98158=EDGE_CURVE ( 'NONE', #47149, #114968, #92797, .T. ) ;
#98159=ORIENTED_EDGE ( 'NONE', *, *, #118438, .F. ) ;
#98160=CIRCLE ( 'NONE', #12187, 0.09999999999999982514 ) ;
#98161=DIRECTION ( 'NONE',  ( 0.000000000000000000, 0.000000000000000000, 1.000000000000000000 ) ) ;
#98162=EDGE_LOOP ( 'NONE', ( #93649, #66336, #39558, #48578 ) ) ;
#98164=DIRECTION ( 'NONE',  ( 0.000000000000000000, -0.000000000000000000, 1.000000000000000000 ) ) ;
#98165=ADVANCED_FACE ( 'NONE', ( #53516 ), #51586, .T. ) ;
#98167=CARTESIAN_POINT ( 'NONE',  ( -4.400000000000025224, 2.500000000000000000, 4.083716857408420609 ) ) ;
#98168=ADVANCED_FACE ( 'NONE', ( #63319 ), #59877, .T. ) ;
#98169=FACE_BOUND ( 'NONE', #19532, .T. ) ;
#98170=EDGE_CURVE ( 'NONE', #120218, #47149, #51544, .T. ) ;
#98171=CARTESIAN_POINT ( 'NONE',  ( -3.100000000000028955, 12.50000000000000000, 4.676537180435972552 ) ) ;
#98172=DIRECTION ( 'NONE',  ( -0.000000000000000000, 1.000000000000000000, -0.000000000000000000 ) ) ;
#98173=DIRECTION ( 'NONE',  ( 0.000000000000000000, 1.000000000000000000, 0.000000000000000000 ) ) ;
#98174=AXIS2_PLACEMENT_3D ( 'NONE', #29105, #19921, #88650 ) ;
#98176=ORIENTED_EDGE ( 'NONE', *, *, #124974, .F. ) ;
#98177=CARTESIAN_POINT ( 'NONE',  ( -14.99999999999998401, 2.500000000000000000, 0.6928203230275518099 ) ) ;
#98178=DIRECTION ( 'NONE',  ( 0.000000000000000000, 0.000000000000000000, 1.000000000000000000 ) ) ;
#98179=EDGE_CURVE ( 'NONE', #14963, #44951, #122550, .T. ) ;
#98180=CARTESIAN_POINT ( 'NONE',  ( 11.04999999999991189, 12.50000000000000000, -2.511473670974877948 ) ) ;
#98182=ORIENTED_EDGE ( 'NONE', *, *, #84990, .F. ) ;
#98183=CIRCLE ( 'NONE', #83627, 0.06509327318403743123 ) ;
#98184=DIRECTION ( 'NONE',  ( 0.000000000000000000, 1.000000000000000000, 0.000000000000000000 ) ) ;
#98185=EDGE_CURVE ( 'NONE', #111368, #22839, #128924, .T. ) ;
#98186=EDGE_CURVE ( 'NONE', #12644, #24551, #91241, .T. ) ;
#98187=CARTESIAN_POINT ( 'NONE',  ( 5.649999999999936406, 2.500000000000000000, -6.148780366869526226 ) ) ;
#98188=AXIS2_PLACEMENT_3D ( 'NONE', #120627, #48673, #79431 ) ;
#98189=VERTEX_POINT ( 'NONE', #113719 ) ;
#98190=ORIENTED_EDGE ( 'NONE', *, *, #117521, .F. ) ;
#98191=CARTESIAN_POINT ( 'NONE',  ( 4.549999999999939426, 2.500000000000000000, -6.495190528383302464 ) ) ;
#98192=DIRECTION ( 'NONE',  ( 0.000000000000000000, -0.000000000000000000, 1.000000000000000000 ) ) ;
#98193=FACE_BOUND ( 'NONE', #96955, .T. ) ;
#98194=ADVANCED_FACE ( 'NONE', ( #122258 ), #11812, .T. ) ;
#98195=CARTESIAN_POINT ( 'NONE',  ( 11.44999999999990692, 12.50000000000000000, -6.841600689897078702 ) ) ;
#98196=EDGE_LOOP ( 'NONE', ( #26292, #27094 ) ) ;
#98197=DIRECTION ( 'NONE',  ( 0.000000000000000000, 1.000000000000000000, 0.000000000000000000 ) ) ;
#98199=ORIENTED_EDGE ( 'NONE', *, *, #44391, .F. ) ;
#98202=EDGE_LOOP ( 'NONE', ( #69908, #77875 ) ) ;
#98203=CARTESIAN_POINT ( 'NONE',  ( 0.6499999999999566125, 2.500000000000000000, -6.941600689897077459 ) ) ;
#98205=PLANE ( 'NONE',  #44262 ) ;
#98206=AXIS2_PLACEMENT_3D ( 'NONE', #125602, #16287, #115795 ) ;
#98207=LINE ( 'NONE', #9834, #84440 ) ;
#98208=ORIENTED_EDGE ( 'NONE', *, *, #60773, .T. ) ;
#98209=DIRECTION ( 'NONE',  ( 0.000000000000000000, 0.000000000000000000, -1.000000000000000000 ) ) ;
#98210=CIRCLE ( 'NONE', #33403, 0.1000000000000002554 ) ;
#98211=CONICAL_SURFACE ( 'NONE', #12, 0.1000000000000002554, 0.003490658503988666988 ) ;
#98212=DIRECTION ( 'NONE',  ( 0.000000000000000000, 0.000000000000000000, 1.000000000000000000 ) ) ;
#98213=CARTESIAN_POINT ( 'NONE',  ( 1.249999999999952038, 2.500000000000000000, -1.572243186433550211 ) ) ;
#98214=CARTESIAN_POINT ( 'NONE',  ( 21.25104878433765876, -0.2455272941117648267, -4.189300629080492833 ) ) ;
#98215=ORIENTED_EDGE ( 'NONE', *, *, #108251, .T. ) ;
#98216=DIRECTION ( 'NONE',  ( 0.000000000000000000, 0.000000000000000000, 1.000000000000000000 ) ) ;
#98217=VERTEX_POINT ( 'NONE', #112437 ) ;
#98218=DIRECTION ( 'NONE',  ( -0.000000000000000000, 1.000000000000000000, -0.000000000000000000 ) ) ;
#98219=EDGE_LOOP ( 'NONE', ( #30326, #44091, #96423, #84532 ) ) ;
#98220=CARTESIAN_POINT ( 'NONE',  ( -6.250000000000019540, 2.500000000000000000, -2.857883832488653741 ) ) ;
#98221=CIRCLE ( 'NONE', #127486, 0.1000000000000002554 ) ;
#98222=CONICAL_SURFACE ( 'NONE', #41821, 0.09999999999999982514, 0.003490658503988666988 ) ;
#98223=CARTESIAN_POINT ( 'NONE',  ( 17.50000000000000000, -2.499999999999999556, -1.666666666666662300 ) ) ;
#98224=EDGE_CURVE ( 'NONE', #50587, #105674, #36867, .T. ) ;
#98225=DIRECTION ( 'NONE',  ( 0.000000000000000000, -0.9999939076577903929, 0.003490651415223739937 ) ) ;
#98226=DIRECTION ( 'NONE',  ( 0.000000000000000000, 0.000000000000000000, 1.000000000000000000 ) ) ;
#98227=ORIENTED_EDGE ( 'NONE', *, *, #91837, .F. ) ;
#98228=DIRECTION ( 'NONE',  ( 0.000000000000000000, 0.000000000000000000, 1.000000000000000000 ) ) ;
#98229=EDGE_CURVE ( 'NONE', #60288, #26496, #110031, .T. ) ;
#98230=DIRECTION ( 'NONE',  ( -0.000000000000000000, -1.000000000000000000, -0.000000000000000000 ) ) ;
#98231=CARTESIAN_POINT ( 'NONE',  ( 87.50000000000001421, 3.974992050023848922, -6.359987280038160051 ) ) ;
#98233=CARTESIAN_POINT ( 'NONE',  ( -12.89999999999999325, 12.50000000000000000, -3.637306695894647390 ) ) ;
#98235=ORIENTED_EDGE ( 'NONE', *, *, #118658, .F. ) ;
#98236=VERTEX_POINT ( 'NONE', #22137 ) ;
#98237=CARTESIAN_POINT ( 'NONE',  ( -11.84999999999999609, 2.500000000000000000, 6.148780366869520897 ) ) ;
#98238=VERTEX_POINT ( 'NONE', #3757 ) ;
#98239=DIRECTION ( 'NONE',  ( 0.000000000000000000, 1.000000000000000000, 0.000000000000000000 ) ) ;
#98240=EDGE_LOOP ( 'NONE', ( #107904, #79783 ) ) ;
#98241=ORIENTED_EDGE ( 'NONE', *, *, #4366, .F. ) ;
#98242=EDGE_LOOP ( 'NONE', ( #87785, #34241 ) ) ;
#98243=CARTESIAN_POINT ( 'NONE',  ( 87.50000000000001421, 3.974992050023852475, -6.359987280038158275 ) ) ;
#98244=AXIS2_PLACEMENT_3D ( 'NONE', #58828, #8420, #126283 ) ;
#98245=FACE_OUTER_BOUND ( 'NONE', #106301, .T. ) ;
#98246=CIRCLE ( 'NONE', #14607, 0.06509327318403745899 ) ;
#98247=CARTESIAN_POINT ( 'NONE',  ( -10.85000000000000142, 2.500000000000000000, -2.957883832488649833 ) ) ;
#98249=PLANE ( 'NONE',  #59840 ) ;
#98250=DIRECTION ( 'NONE',  ( -4.274815082592931898E-19, -0.9999939076577903929, -0.003490651415223739937 ) ) ;
#98251=DIRECTION ( 'NONE',  ( 0.000000000000000000, 0.000000000000000000, 1.000000000000000000 ) ) ;
#98252=DIRECTION ( 'NONE',  ( -4.274815082592931898E-19, -0.9999939076577903929, -0.003490651415223739937 ) ) ;
#98253=DIRECTION ( 'NONE',  ( -0.000000000000000000, -1.000000000000000000, -0.000000000000000000 ) ) ;
#98254=CONICAL_SURFACE ( 'NONE', #31379, 0.1000000000000002554, 0.003490658503988666988 ) ;
#98255=ORIENTED_EDGE ( 'NONE', *, *, #3023, .F. ) ;
#98256=VERTEX_POINT ( 'NONE', #83621 ) ;
#98257=ORIENTED_EDGE ( 'NONE', *, *, #19568, .T. ) ;
#98258=FACE_OUTER_BOUND ( 'NONE', #14777, .T. ) ;
#98259=EDGE_LOOP ( 'NONE', ( #11543, #59495, #9244, #73292 ) ) ;
#98260=ORIENTED_EDGE ( 'NONE', *, *, #16995, .T. ) ;
#98261=DIRECTION ( 'NONE',  ( 0.000000000000000000, -0.9999939076577903929, 0.003490651415223739937 ) ) ;
#98262=CIRCLE ( 'NONE', #41854, 0.06509327318403745899 ) ;
#98263=VECTOR ( 'NONE', #29571, 1000.000000000000000 ) ;
#98264=EDGE_CURVE ( 'NONE', #55968, #107226, #68240, .T. ) ;
#98265=DIRECTION ( 'NONE',  ( -0.000000000000000000, 1.000000000000000000, -0.000000000000000000 ) ) ;
#98266=DIRECTION ( 'NONE',  ( 0.000000000000000000, 0.000000000000000000, 1.000000000000000000 ) ) ;
#98267=CIRCLE ( 'NONE', #41859, 0.1000000000000002554 ) ;
#98268=FACE_OUTER_BOUND ( 'NONE', #27225, .T. ) ;
#98269=PLANE ( 'NONE',  #99430 ) ;
#98270=DIRECTION ( 'NONE',  ( 0.000000000000000000, 0.000000000000000000, 1.000000000000000000 ) ) ;
#98271=ORIENTED_EDGE ( 'NONE', *, *, #127003, .T. ) ;
#98272=CARTESIAN_POINT ( 'NONE',  ( -11.69999999999999574, 2.500000000000000000, 4.330127018922196314 ) ) ;
#98273=ORIENTED_EDGE ( 'NONE', *, *, #102788, .T. ) ;
#98274=CARTESIAN_POINT ( 'NONE',  ( -11.44999999999999751, 2.500000000000000000, -6.841600689897074261 ) ) ;
#98275=VERTEX_POINT ( 'NONE', #11644 ) ;
#98276=DIRECTION ( 'NONE',  ( -0.000000000000000000, 1.000000000000000000, -0.000000000000000000 ) ) ;
#98277=AXIS2_PLACEMENT_3D ( 'NONE', #21573, #121056, #49766 ) ;
#98278=ORIENTED_EDGE ( 'NONE', *, *, #8145, .T. ) ;
#98279=EDGE_CURVE ( 'NONE', #35495, #20160, #2448, .T. ) ;
#98280=EDGE_CURVE ( 'NONE', #25512, #11963, #62049, .T. ) ;
#98281=EDGE_LOOP ( 'NONE', ( #31827, #57812 ) ) ;
#98282=CARTESIAN_POINT ( 'NONE',  ( 7.499999999999927169, 12.50000000000000000, -5.088040615133791356 ) ) ;
#98283=CARTESIAN_POINT ( 'NONE',  ( -12.49999999999995914, 12.50000000000000000, 1.843143693225357538E-15 ) ) ;
#98284=CARTESIAN_POINT ( 'NONE',  ( -6.850000000000013856, 2.500000000000000000, 2.511473670974873507 ) ) ;
#98285=DIRECTION ( 'NONE',  ( 0.000000000000000000, 0.000000000000000000, 1.000000000000000000 ) ) ;
#98286=FACE_OUTER_BOUND ( 'NONE', #11061, .T. ) ;
#98287=VERTEX_POINT ( 'NONE', #22777 ) ;
#98288=PLANE ( 'NONE',  #108465 ) ;
#98289=CARTESIAN_POINT ( 'NONE',  ( 9.599999999999914380, 2.500000000000000000, -4.330127018922201643 ) ) ;
#98290=ADVANCED_FACE ( 'NONE', ( #62693 ), #103766, .T. ) ;
#98291=DIRECTION ( 'NONE',  ( 0.000000000000000000, 0.000000000000000000, 1.000000000000000000 ) ) ;
#98292=CARTESIAN_POINT ( 'NONE',  ( 12.49999999999993960, 12.50000000000000000, 4.330127018922196314 ) ) ;
#98293=FACE_OUTER_BOUND ( 'NONE', #117900, .T. ) ;
#98294=VERTEX_POINT ( 'NONE', #24695 ) ;
#98295=VERTEX_POINT ( 'NONE', #116917 ) ;
#98296=AXIS2_PLACEMENT_3D ( 'NONE', #28565, #39055, #109709 ) ;
#98297=DIRECTION ( 'NONE',  ( -0.000000000000000000, -1.000000000000000000, -0.000000000000000000 ) ) ;
#98298=CONICAL_SURFACE ( 'NONE', #119237, 0.1000000000000002554, 0.003490658503988666988 ) ;
#98299=ORIENTED_EDGE ( 'NONE', *, *, #6502, .F. ) ;
#98300=LINE ( 'NONE', #9291, #19481 ) ;
#98301=CARTESIAN_POINT ( 'NONE',  ( -5.650000000000019895, 2.500000000000000000, 2.511473670974873507 ) ) ;
#98302=AXIS2_PLACEMENT_3D ( 'NONE', #15224, #53889, #93817 ) ;
#98303=AXIS2_PLACEMENT_3D ( 'NONE', #8827, #48783, #69049 ) ;
#98304=ORIENTED_EDGE ( 'NONE', *, *, #108839, .T. ) ;
#98306=DIRECTION ( 'NONE',  ( 0.000000000000000000, -0.000000000000000000, 1.000000000000000000 ) ) ;
#98307=CARTESIAN_POINT ( 'NONE',  ( -4.550000000000022915, 12.50000000000000000, 2.099970236277060032 ) ) ;
#98308=CARTESIAN_POINT ( 'NONE',  ( 13.09999999999989839, 12.50000000000000000, -0.3464101615137783474 ) ) ;
#98309=ORIENTED_EDGE ( 'NONE', *, *, #45695, .T. ) ;
#98310=EDGE_CURVE ( 'NONE', #98275, #57844, #87029, .T. ) ;
#98311=CARTESIAN_POINT ( 'NONE',  ( 3.749999999999944045, 12.50000000000000000, -7.188010851410854052 ) ) ;
#98312=EDGE_LOOP ( 'NONE', ( #4820, #15148 ) ) ;
#98313=EDGE_CURVE ( 'NONE', #62529, #95423, #118423, .T. ) ;
#98314=CARTESIAN_POINT ( 'NONE',  ( 34.93098733902322550, 2.900247951333832841, -4.640741454330529869 ) ) ;
#98315=CARTESIAN_POINT ( 'NONE',  ( -2.500000000000032419, 2.500000000000000000, 0.6928203230275494784 ) ) ;
#98316=ADVANCED_FACE ( 'NONE', ( #66535 ), #104535, .T. ) ;
#98317=CARTESIAN_POINT ( 'NONE',  ( 2.899999999999945732, 2.500000000000000000, -4.230127018922201998 ) ) ;
#98318=EDGE_LOOP ( 'NONE', ( #128474, #117712, #18976, #96493 ) ) ;
#98319=CARTESIAN_POINT ( 'NONE',  ( -3.100000000000028511, 2.500000000000000000, -0.3464101615137782364 ) ) ;
#98320=EDGE_CURVE ( 'NONE', #67065, #114454, #59972, .T. ) ;
#98321=EDGE_CURVE ( 'NONE', #36118, #9409, #96007, .T. ) ;
#98322=EDGE_LOOP ( 'NONE', ( #84814, #52564, #58473, #50559 ) ) ;
#98323=CARTESIAN_POINT ( 'NONE',  ( 9.149999999999918643, 12.50000000000000000, 2.165063509461097713 ) ) ;
#98324=LINE ( 'NONE', #118619, #98978 ) ;
#98325=EDGE_CURVE ( 'NONE', #70057, #41901, #57899, .T. ) ;
#98326=EDGE_CURVE ( 'NONE', #1374, #4680, #30721, .T. ) ;
#98327=FACE_OUTER_BOUND ( 'NONE', #45998, .T. ) ;
#98328=ORIENTED_EDGE ( 'NONE', *, *, #46913, .F. ) ;
#98329=AXIS2_PLACEMENT_3D ( 'NONE', #127125, #47917, #77371 ) ;
#98330=FACE_OUTER_BOUND ( 'NONE', #13978, .T. ) ;
#98331=VECTOR ( 'NONE', #124840, 1000.000000000000000 ) ;
#98332=EDGE_CURVE ( 'NONE', #78481, #120522, #6308, .T. ) ;
#98333=CARTESIAN_POINT ( 'NONE',  ( -4.200000000000025935, 2.500000000000000000, -2.385244779468109755E-15 ) ) ;
#98334=ORIENTED_EDGE ( 'NONE', *, *, #77364, .F. ) ;
#98335=CARTESIAN_POINT ( 'NONE',  ( -0.8500000000000386136, 2.500000000000000000, 7.288010851410849256 ) ) ;
#98336=EDGE_LOOP ( 'NONE', ( #53808, #24121, #96979, #13237 ) ) ;
#98337=EDGE_CURVE ( 'NONE', #45239, #110014, #17739, .T. ) ;
#98338=DIRECTION ( 'NONE',  ( -0.000000000000000000, 1.000000000000000000, -0.000000000000000000 ) ) ;
#98339=EDGE_LOOP ( 'NONE', ( #23011, #2795 ) ) ;
#98341=DIRECTION ( 'NONE',  ( 0.000000000000000000, 1.000000000000000000, 0.000000000000000000 ) ) ;
#98342=ORIENTED_EDGE ( 'NONE', *, *, #8458, .F. ) ;
#98343=VERTEX_POINT ( 'NONE', #25310 ) ;
#98344=DIRECTION ( 'NONE',  ( 0.000000000000000000, 1.000000000000000000, 0.000000000000000000 ) ) ;
#98345=FACE_OUTER_BOUND ( 'NONE', #7383, .T. ) ;
#98346=ORIENTED_EDGE ( 'NONE', *, *, #121851, .F. ) ;
#98347=AXIS2_PLACEMENT_3D ( 'NONE', #38780, #110074, #21040 ) ;
#98350=AXIS2_PLACEMENT_3D ( 'NONE', #73231, #78714, #118616 ) ;
#98351=DIRECTION ( 'NONE',  ( 0.000000000000000000, 1.000000000000000000, 0.000000000000000000 ) ) ;
#98352=DIRECTION ( 'NONE',  ( 0.000000000000000000, 0.000000000000000000, 1.000000000000000000 ) ) ;
#98353=CARTESIAN_POINT ( 'NONE',  ( -2.100000000000034284, 12.50000000000000000, -4.330127018922201643 ) ) ;
#98354=DIRECTION ( 'NONE',  ( -0.000000000000000000, -1.000000000000000000, -0.000000000000000000 ) ) ;
#98355=DIRECTION ( 'NONE',  ( 0.000000000000000000, 0.000000000000000000, 1.000000000000000000 ) ) ;
#98356=CONICAL_SURFACE ( 'NONE', #56587, 0.1000000000000002554, 0.003490658503988666988 ) ;
#98357=ORIENTED_EDGE ( 'NONE', *, *, #22308, .T. ) ;
#98358=EDGE_LOOP ( 'NONE', ( #115098, #126346 ) ) ;
#98359=VERTEX_POINT ( 'NONE', #126765 ) ;
#98360=VERTEX_POINT ( 'NONE', #124178 ) ;
#98362=CARTESIAN_POINT ( 'NONE',  ( 0.1999999999999627909, 12.50000000000000000, 0.3464101615137758494 ) ) ;
#98363=CARTESIAN_POINT ( 'NONE',  ( 10.84999999999990905, 12.50000000000000000, 2.165063509461097713 ) ) ;
#98364=DIRECTION ( 'NONE',  ( 0.000000000000000000, 0.000000000000000000, 1.000000000000000000 ) ) ;
#98365=ORIENTED_EDGE ( 'NONE', *, *, #21835, .F. ) ;
#98366=FACE_BOUND ( 'NONE', #127118, .T. ) ;
#98367=ORIENTED_EDGE ( 'NONE', *, *, #4222, .F. ) ;
#98368=FACE_OUTER_BOUND ( 'NONE', #3654, .T. ) ;
#98369=DIRECTION ( 'NONE',  ( 0.000000000000000000, 0.000000000000000000, 1.000000000000000000 ) ) ;
#98370=DIRECTION ( 'NONE',  ( 0.000000000000000000, -0.9999939076577903929, 0.003490651415223739937 ) ) ;
#98371=EDGE_CURVE ( 'NONE', #75848, #125178, #112273, .T. ) ;
#98372=CARTESIAN_POINT ( 'NONE',  ( -10.65000000000000213, 2.500000000000000000, 6.841600689897072485 ) ) ;
#98373=DIRECTION ( 'NONE',  ( -4.274815082592931898E-19, -0.9999939076577903929, -0.003490651415223739937 ) ) ;
#98374=CARTESIAN_POINT ( 'NONE',  ( 10.84999999999990905, 12.50000000000000000, -5.802370205355749988 ) ) ;
#98375=CARTESIAN_POINT ( 'NONE',  ( -4.600000000000024514, 12.50000000000000000, -0.6928203230275542523 ) ) ;
#98376=DIRECTION ( 'NONE',  ( 0.000000000000000000, 1.000000000000000000, 0.000000000000000000 ) ) ;
#98377=DIRECTION ( 'NONE',  ( -0.000000000000000000, -1.000000000000000000, -0.000000000000000000 ) ) ;
#98378=DIRECTION ( 'NONE',  ( 0.000000000000000000, 0.000000000000000000, 1.000000000000000000 ) ) ;
#98379=EDGE_CURVE ( 'NONE', #106850, #35030, #76666, .T. ) ;
#98380=ORIENTED_EDGE ( 'NONE', *, *, #78900, .T. ) ;
#98381=ORIENTED_EDGE ( 'NONE', *, *, #76038, .T. ) ;
#98382=VERTEX_POINT ( 'NONE', #76374 ) ;
#98383=VERTEX_POINT ( 'NONE', #75706 ) ;
#98384=DIRECTION ( 'NONE',  ( -0.000000000000000000, -1.000000000000000000, -0.000000000000000000 ) ) ;
#98385=AXIS2_PLACEMENT_3D ( 'NONE', #19722, #118550, #110663 ) ;
#98386=CARTESIAN_POINT ( 'NONE',  ( 4.799999999999939426, 2.500000000000000000, -4.576537180435977348 ) ) ;
#98387=AXIS2_PLACEMENT_3D ( 'NONE', #2820, #63032, #83329 ) ;
#98388=CIRCLE ( 'NONE', #2239, 0.06509327318403741736 ) ;
#98389=ORIENTED_EDGE ( 'NONE', *, *, #124892, .T. ) ;
#98390=ORIENTED_EDGE ( 'NONE', *, *, #117956, .F. ) ;
#98391=EDGE_LOOP ( 'NONE', ( #51977, #10599, #64401, #99210 ) ) ;
#98392=DIRECTION ( 'NONE',  ( 0.000000000000000000, 1.000000000000000000, 0.000000000000000000 ) ) ;
#98393=AXIS2_PLACEMENT_3D ( 'NONE', #110, #61632, #89788 ) ;
#98394=DIRECTION ( 'NONE',  ( -0.000000000000000000, -1.000000000000000000, -0.000000000000000000 ) ) ;
#98395=CARTESIAN_POINT ( 'NONE',  ( -1.050000000000038680, 2.500000000000000000, 2.411473670974873862 ) ) ;
#98396=CARTESIAN_POINT ( 'NONE',  ( -10.20000000000000462, 12.50000000000000000, 0.3464101615137735735 ) ) ;
#98397=CARTESIAN_POINT ( 'NONE',  ( 11.44999999999990514, 2.500000000000000000, 2.511473670974873507 ) ) ;
#98398=DIRECTION ( 'NONE',  ( 0.000000000000000000, 0.000000000000000000, 1.000000000000000000 ) ) ;
#98399=CIRCLE ( 'NONE', #73359, 0.06509327318403745899 ) ;
#98400=DIRECTION ( 'NONE',  ( 0.000000000000000000, 0.000000000000000000, 1.000000000000000000 ) ) ;
#98401=EDGE_LOOP ( 'NONE', ( #107478, #3733 ) ) ;
#98402=CARTESIAN_POINT ( 'NONE',  ( 6.249999999999930722, 12.50000000000000000, 1.472243186433545459 ) ) ;
#98403=ORIENTED_EDGE ( 'NONE', *, *, #109078, .F. ) ;
#98404=VERTEX_POINT ( 'NONE', #15498 ) ;
#98405=VERTEX_POINT ( 'NONE', #34530 ) ;
#98406=CARTESIAN_POINT ( 'NONE',  ( -0.8500000000000386136, 2.500000000000000000, 7.188010851410848723 ) ) ;
#98407=EDGE_LOOP ( 'NONE', ( #118743, #16775 ) ) ;
#98408=ORIENTED_EDGE ( 'NONE', *, *, #87631, .F. ) ;
#98409=DIRECTION ( 'NONE',  ( 0.000000000000000000, 0.000000000000000000, -1.000000000000000000 ) ) ;
#98410=EDGE_CURVE ( 'NONE', #115296, #115890, #5671, .T. ) ;
#98411=DIRECTION ( 'NONE',  ( -0.000000000000000000, 1.000000000000000000, -0.000000000000000000 ) ) ;
#98412=DIRECTION ( 'NONE',  ( 0.000000000000000000, -0.000000000000000000, 1.000000000000000000 ) ) ;
#98413=DIRECTION ( 'NONE',  ( 0.000000000000000000, 1.000000000000000000, 0.000000000000000000 ) ) ;
#98415=VERTEX_POINT ( 'NONE', #26622 ) ;
#98416=FACE_OUTER_BOUND ( 'NONE', #100733, .T. ) ;
#98417=VECTOR ( 'NONE', #99593, 1000.000000000000000 ) ;
#98418=EDGE_CURVE ( 'NONE', #93494, #4249, #129014, .T. ) ;
#98419=CIRCLE ( 'NONE', #58733, 0.1000000000000000472 ) ;
#98420=VERTEX_POINT ( 'NONE', #16772 ) ;
#98421=DIRECTION ( 'NONE',  ( 0.000000000000000000, -0.000000000000000000, 1.000000000000000000 ) ) ;
#98422=VERTEX_POINT ( 'NONE', #56696 ) ;
#98424=FACE_OUTER_BOUND ( 'NONE', #46029, .T. ) ;
#98425=ORIENTED_EDGE ( 'NONE', *, *, #83752, .T. ) ;
#98426=CARTESIAN_POINT ( 'NONE',  ( 8.099999999999923261, 2.500000000000000000, -4.676537180435978769 ) ) ;
#98427=ADVANCED_FACE ( 'NONE', ( #6947 ), #46920, .T. ) ;
#98428=CARTESIAN_POINT ( 'NONE',  ( 1.249999999999954259, 12.50000000000000000, -7.253104124594891289 ) ) ;
#98429=ADVANCED_FACE ( 'NONE', ( #9564 ), #93390, .T. ) ;
#98430=ORIENTED_EDGE ( 'NONE', *, *, #51288, .T. ) ;
#98431=AXIS2_PLACEMENT_3D ( 'NONE', #91194, #101668, #882 ) ;
#98433=EDGE_CURVE ( 'NONE', #92053, #76876, #7688, .T. ) ;
#98434=DIRECTION ( 'NONE',  ( 0.000000000000000000, 1.000000000000000000, 0.000000000000000000 ) ) ;
#98435=ORIENTED_EDGE ( 'NONE', *, *, #127581, .T. ) ;
#98436=ORIENTED_EDGE ( 'NONE', *, *, #11897, .F. ) ;
#98437=CARTESIAN_POINT ( 'NONE',  ( -0.4000000000000401013, 2.500000000000000000, -3.637306695894650055 ) ) ;
#98438=DIRECTION ( 'NONE',  ( 0.000000000000000000, 1.000000000000000000, 0.000000000000000000 ) ) ;
#98439=EDGE_CURVE ( 'NONE', #110749, #74045, #74607, .T. ) ;
#98441=CARTESIAN_POINT ( 'NONE',  ( 0.1999999999999562961, 2.500000000000000000, 4.576537180435972019 ) ) ;
#98442=AXIS2_PLACEMENT_3D ( 'NONE', #122328, #92195, #103322 ) ;
#98443=VECTOR ( 'NONE', #17513, 1000.000000000000000 ) ;
#98445=ORIENTED_EDGE ( 'NONE', *, *, #62514, .T. ) ;
#98446=CARTESIAN_POINT ( 'NONE',  ( -10.20000000000000284, 2.500000000000000000, 3.983716857408420964 ) ) ;
#98447=AXIS2_PLACEMENT_3D ( 'NONE', #118306, #127494, #59416 ) ;
#98449=DIRECTION ( 'NONE',  ( 0.000000000000000000, 1.000000000000000000, 0.000000000000000000 ) ) ;
#98450=DIRECTION ( 'NONE',  ( -0.000000000000000000, -1.000000000000000000, -0.000000000000000000 ) ) ;
#98451=VERTEX_POINT ( 'NONE', #109704 ) ;
#98452=CIRCLE ( 'NONE', #39998, 0.06509327318403745899 ) ;
#98453=CARTESIAN_POINT ( 'NONE',  ( -11.24999999999996447, 2.500000000000000000, -2.265063509461097802 ) ) ;
#98454=DIRECTION ( 'NONE',  ( -4.274815082592931898E-19, -0.9999939076577903929, -0.003490651415223739937 ) ) ;
#98455=DIRECTION ( 'NONE',  ( -0.000000000000000000, -1.000000000000000000, -0.000000000000000000 ) ) ;
#98457=CARTESIAN_POINT ( 'NONE',  ( 0.1999999999999567124, 12.50000000000000000, -3.918623584224389056 ) ) ;
#98458=ORIENTED_EDGE ( 'NONE', *, *, #22168, .F. ) ;
#98459=CARTESIAN_POINT ( 'NONE',  ( 2.899999999999945732, 2.500000000000000000, -2.385244779468109755E-15 ) ) ;
#98460=DIRECTION ( 'NONE',  ( 0.000000000000000000, 0.000000000000000000, -1.000000000000000000 ) ) ;
#98461=ORIENTED_EDGE ( 'NONE', *, *, #72394, .T. ) ;
#98462=ADVANCED_FACE ( 'NONE', ( #107758 ), #78320, .T. ) ;
#98463=CARTESIAN_POINT ( 'NONE',  ( -4.350000000000023626, 2.500000000000000000, 6.148780366869520897 ) ) ;
#98464=ORIENTED_EDGE ( 'NONE', *, *, #17150, .F. ) ;
#98465=EDGE_LOOP ( 'NONE', ( #29425, #54374, #98389, #13997 ) ) ;
#98466=DIRECTION ( 'NONE',  ( -0.000000000000000000, -1.000000000000000000, -0.000000000000000000 ) ) ;
#98467=CONICAL_SURFACE ( 'NONE', #73441, 0.1000000000000002554, 0.003490658503988666988 ) ;
#98468=EDGE_CURVE ( 'NONE', #80552, #93103, #99649, .T. ) ;
#98469=AXIS2_PLACEMENT_3D ( 'NONE', #11184, #10535, #90379 ) ;
#98470=EDGE_CURVE ( 'NONE', #67325, #124086, #99242, .T. ) ;
#98471=CONICAL_SURFACE ( 'NONE', #115185, 0.1000000000000002554, 0.003490658503988666988 ) ;
#98473=DIRECTION ( 'NONE',  ( 0.000000000000000000, 1.000000000000000000, 0.000000000000000000 ) ) ;
#98474=CARTESIAN_POINT ( 'NONE',  ( 1.849999999999951017, 2.500000000000000000, -6.148780366869526226 ) ) ;
#98475=EDGE_CURVE ( 'NONE', #23121, #103499, #89277, .T. ) ;
#98476=EDGE_CURVE ( 'NONE', #32813, #76857, #39131, .T. ) ;
#98477=VERTEX_POINT ( 'NONE', #19360 ) ;
#98478=CIRCLE ( 'NONE', #115188, 0.06509327318403745899 ) ;
#98479=DIRECTION ( 'NONE',  ( -0.000000000000000000, 1.000000000000000000, -0.000000000000000000 ) ) ;
#98480=EDGE_CURVE ( 'NONE', #35232, #13086, #49496, .T. ) ;
#98481=CARTESIAN_POINT ( 'NONE',  ( -9.150000000000009237, 12.50000000000000000, 1.472243186433545459 ) ) ;
#98482=ORIENTED_EDGE ( 'NONE', *, *, #39373, .F. ) ;
#98483=VECTOR ( 'NONE', #68308, 1000.000000000000000 ) ;
#98484=DIRECTION ( 'NONE',  ( 0.000000000000000000, 0.000000000000000000, 1.000000000000000000 ) ) ;
#98485=CARTESIAN_POINT ( 'NONE',  ( 7.899999999999924860, 12.50000000000000000, 4.265033745738159077 ) ) ;
#98486=ORIENTED_EDGE ( 'NONE', *, *, #32015, .T. ) ;
#98487=EDGE_CURVE ( 'NONE', #88341, #19578, #20677, .T. ) ;
#98489=VERTEX_POINT ( 'NONE', #118868 ) ;
#98491=DIRECTION ( 'NONE',  ( 0.000000000000000000, -0.000000000000000000, 1.000000000000000000 ) ) ;
#98492=CARTESIAN_POINT ( 'NONE',  ( 13.09999999999990195, 2.500000000000000000, 3.983716857408420076 ) ) ;
#98493=DIRECTION ( 'NONE',  ( -0.000000000000000000, 1.000000000000000000, -0.000000000000000000 ) ) ;
#98494=FACE_BOUND ( 'NONE', #10263, .T. ) ;
#98495=EDGE_LOOP ( 'NONE', ( #17531, #8912, #54067, #107761 ) ) ;
#98496=FACE_OUTER_BOUND ( 'NONE', #96354, .T. ) ;
#98497=LINE ( 'NONE', #10141, #119242 ) ;
#98498=ORIENTED_EDGE ( 'NONE', *, *, #102441, .F. ) ;
#98500=CARTESIAN_POINT ( 'NONE',  ( 5.849999999999933920, 12.50000000000000000, 6.560283801567334372 ) ) ;
#98501=DIRECTION ( 'NONE',  ( 0.000000000000000000, 1.000000000000000000, 0.000000000000000000 ) ) ;
#98502=CARTESIAN_POINT ( 'NONE',  ( -13.14999999999999147, 2.500000000000000000, 2.611473670974877148 ) ) ;
#98503=CARTESIAN_POINT ( 'NONE',  ( -12.29999999999999538, 2.500000000000000000, 4.676537180435972552 ) ) ;
#98504=CARTESIAN_POINT ( 'NONE',  ( 12.04999999999990834, 12.50000000000000000, 6.430097255199259010 ) ) ;
#98505=CARTESIAN_POINT ( 'NONE',  ( -9.550000000000007816, 2.500000000000000000, -6.495190528383297135 ) ) ;
#98506=VECTOR ( 'NONE', #102785, 1000.000000000000000 ) ;
#98507=ORIENTED_EDGE ( 'NONE', *, *, #57298, .T. ) ;
#98508=VERTEX_POINT ( 'NONE', #58668 ) ;
#98509=ORIENTED_EDGE ( 'NONE', *, *, #104536, .T. ) ;
#98511=EDGE_LOOP ( 'NONE', ( #32496, #93974, #117631, #46767 ) ) ;
#98512=DIRECTION ( 'NONE',  ( 0.000000000000000000, 1.000000000000000000, 0.000000000000000000 ) ) ;
#98513=FACE_OUTER_BOUND ( 'NONE', #1186, .T. ) ;
#98514=EDGE_LOOP ( 'NONE', ( #44890, #128454 ) ) ;
#98515=FACE_BOUND ( 'NONE', #90376, .T. ) ;
#98516=AXIS2_PLACEMENT_3D ( 'NONE', #8480, #48421, #88322 ) ;
#98517=FACE_OUTER_BOUND ( 'NONE', #57379, .T. ) ;
#98518=CIRCLE ( 'NONE', #108984, 0.09999999999999982514 ) ;
#98519=DIRECTION ( 'NONE',  ( 0.000000000000000000, -0.9999939076577903929, 0.003490651415223739937 ) ) ;
#98520=DIRECTION ( 'NONE',  ( 0.000000000000000000, 1.000000000000000000, 0.000000000000000000 ) ) ;
#98521=CARTESIAN_POINT ( 'NONE',  ( 8.349999999999919709, 2.500000000000000000, 6.495190528383297135 ) ) ;
#98522=FACE_OUTER_BOUND ( 'NONE', #100512, .T. ) ;
#98523=ORIENTED_EDGE ( 'NONE', *, *, #33005, .F. ) ;
#98524=AXIS2_PLACEMENT_3D ( 'NONE', #80951, #120228, #22040 ) ;
#98525=ORIENTED_EDGE ( 'NONE', *, *, #126524, .T. ) ;
#98527=ORIENTED_EDGE ( 'NONE', *, *, #90607, .T. ) ;
#98528=VERTEX_POINT ( 'NONE', #8897 ) ;
#98529=VECTOR ( 'NONE', #60024, 1000.000000000000000 ) ;
#98530=DIRECTION ( 'NONE',  ( 0.000000000000000000, -0.000000000000000000, 1.000000000000000000 ) ) ;
#98531=CARTESIAN_POINT ( 'NONE',  ( 8.340322510150830482, 2.500000000000000000, 8.517653998215561018 ) ) ;
#98532=DIRECTION ( 'NONE',  ( 0.000000000000000000, 0.000000000000000000, 1.000000000000000000 ) ) ;
#98533=EDGE_LOOP ( 'NONE', ( #11361, #75752, #70086, #115181 ) ) ;
#98534=DIRECTION ( 'NONE',  ( 0.000000000000000000, 1.000000000000000000, 0.000000000000000000 ) ) ;
#98535=CIRCLE ( 'NONE', #123584, 0.1000000000000002554 ) ;
#98536=PLANE ( 'NONE',  #105490 ) ;
#98537=DIRECTION ( 'NONE',  ( -0.000000000000000000, -1.000000000000000000, -0.000000000000000000 ) ) ;
#98538=AXIS2_PLACEMENT_3D ( 'NONE', #19821, #27679, #68256 ) ;
#98539=AXIS2_PLACEMENT_3D ( 'NONE', #126775, #36478, #128061 ) ;
#98541=DIRECTION ( 'NONE',  ( 0.000000000000000000, 0.000000000000000000, -1.000000000000000000 ) ) ;
#98542=CARTESIAN_POINT ( 'NONE',  ( 13.29999999999990301, 12.50000000000000000, 4.265033745738159077 ) ) ;
#98543=DIRECTION ( 'NONE',  ( 0.000000000000000000, 1.000000000000000000, 0.000000000000000000 ) ) ;
#98545=DIRECTION ( 'NONE',  ( -4.274815082592931898E-19, -0.9999939076577903929, -0.003490651415223739937 ) ) ;
#98546=VERTEX_POINT ( 'NONE', #8257 ) ;
#98547=ORIENTED_EDGE ( 'NONE', *, *, #105933, .T. ) ;
#98548=CARTESIAN_POINT ( 'NONE',  ( 5.399999999999935518, 12.50000000000000000, -4.330127018922201643 ) ) ;
#98549=LINE ( 'NONE', #88758, #69867 ) ;
#98550=CARTESIAN_POINT ( 'NONE',  ( -2.100000000000033396, 2.500000000000000000, -0.7928203230275543412 ) ) ;
#98551=EDGE_CURVE ( 'NONE', #82416, #64406, #48194, .T. ) ;
#98552=ORIENTED_EDGE ( 'NONE', *, *, #126260, .T. ) ;
#98553=EDGE_LOOP ( 'NONE', ( #68235, #67510, #23648, #84562 ) ) ;
#98554=DIRECTION ( 'NONE',  ( -0.000000000000000000, -1.000000000000000000, -0.000000000000000000 ) ) ;
#98556=CIRCLE ( 'NONE', #61012, 0.06509327318403745899 ) ;
#98557=DIRECTION ( 'NONE',  ( -0.000000000000000000, 1.000000000000000000, -0.000000000000000000 ) ) ;
#98559=ORIENTED_EDGE ( 'NONE', *, *, #63505, .T. ) ;
#98560=AXIS2_PLACEMENT_3D ( 'NONE', #880, #10058, #12616 ) ;
#98562=EDGE_CURVE ( 'NONE', #29366, #48393, #3507, .T. ) ;
#98563=VERTEX_POINT ( 'NONE', #20033 ) ;
#98564=DIRECTION ( 'NONE',  ( -0.000000000000000000, -1.000000000000000000, -0.000000000000000000 ) ) ;
#98565=EDGE_CURVE ( 'NONE', #92934, #128018, #72565, .T. ) ;
#98566=CIRCLE ( 'NONE', #27559, 0.06509327318403745899 ) ;
#98568=DIRECTION ( 'NONE',  ( -4.274815082592931898E-19, -0.9999939076577903929, -0.003490651415223739937 ) ) ;
#98569=CIRCLE ( 'NONE', #44203, 0.06509327318403745899 ) ;
#98570=DIRECTION ( 'NONE',  ( 0.000000000000000000, 0.000000000000000000, 1.000000000000000000 ) ) ;
#98571=CARTESIAN_POINT ( 'NONE',  ( -2.900000000000029221, 12.50000000000000000, -4.330127018922201643 ) ) ;
#98572=VECTOR ( 'NONE', #44292, 1000.000000000000000 ) ;
#98573=ADVANCED_FACE ( 'NONE', ( #50145 ), #16088, .T. ) ;
#98574=DIRECTION ( 'NONE',  ( 0.000000000000000000, 0.000000000000000000, 1.000000000000000000 ) ) ;
#98575=EDGE_CURVE ( 'NONE', #118566, #83964, #70405, .T. ) ;
#98576=VERTEX_POINT ( 'NONE', #71060 ) ;
#98577=AXIS2_PLACEMENT_3D ( 'NONE', #108347, #79546, #116868 ) ;
#98578=DIRECTION ( 'NONE',  ( 0.000000000000000000, 1.000000000000000000, 0.000000000000000000 ) ) ;
#98579=EDGE_CURVE ( 'NONE', #100174, #15903, #97584, .T. ) ;
#98580=VERTEX_POINT ( 'NONE', #63823 ) ;
#98581=ADVANCED_FACE ( 'NONE', ( #33092 ), #122099, .T. ) ;
#98582=ORIENTED_EDGE ( 'NONE', *, *, #237, .T. ) ;
#98583=EDGE_CURVE ( 'NONE', #115200, #76721, #62102, .T. ) ;
#98584=LINE ( 'NONE', #60000, #85214 ) ;
#98585=FACE_OUTER_BOUND ( 'NONE', #30258, .T. ) ;
#98586=CARTESIAN_POINT ( 'NONE',  ( 17.50000000000000000, 2.500000000000000000, 2.922290670087886344 ) ) ;
#98587=ADVANCED_FACE ( 'NONE', ( #52700 ), #103857, .T. ) ;
#98588=DIRECTION ( 'NONE',  ( 0.000000000000000000, 0.000000000000000000, 1.000000000000000000 ) ) ;
#98589=LINE ( 'NONE', #90065, #113897 ) ;
#98590=DIRECTION ( 'NONE',  ( 0.000000000000000000, 0.000000000000000000, 1.000000000000000000 ) ) ;
#98591=CARTESIAN_POINT ( 'NONE',  ( -13.94999999999998863, 2.500000000000000000, -1.818653347947323917 ) ) ;
#98592=DIRECTION ( 'NONE',  ( 0.000000000000000000, 0.000000000000000000, 1.000000000000000000 ) ) ;
#98593=CARTESIAN_POINT ( 'NONE',  ( 6.849999999999929479, 2.500000000000000000, -2.411473670974877859 ) ) ;
#98594=EDGE_CURVE ( 'NONE', #125908, #109519, #13955, .T. ) ;
#98595=DIRECTION ( 'NONE',  ( 0.000000000000000000, -0.000000000000000000, 1.000000000000000000 ) ) ;
#98596=CONICAL_SURFACE ( 'NONE', #106923, 0.1000000000000002554, 0.003490658503988666988 ) ;
#98597=AXIS2_PLACEMENT_3D ( 'NONE', #104241, #76714, #84606 ) ;
#98598=VERTEX_POINT ( 'NONE', #31154 ) ;
#98599=DIRECTION ( 'NONE',  ( 0.000000000000000000, 1.000000000000000000, 0.000000000000000000 ) ) ;
#98600=CARTESIAN_POINT ( 'NONE',  ( 14.34999999999989662, 2.500000000000000000, 1.818653347947321475 ) ) ;
#98601=CARTESIAN_POINT ( 'NONE',  ( 0.8499999999999536815, 12.50000000000000000, 5.802370205355744659 ) ) ;
#98602=DIRECTION ( 'NONE',  ( 0.000000000000000000, 1.000000000000000000, 0.000000000000000000 ) ) ;
#98603=CARTESIAN_POINT ( 'NONE',  ( 1.449999999999950440, 12.50000000000000000, 6.213873640053558134 ) ) ;
#98604=CONICAL_SURFACE ( 'NONE', #90290, 0.1000000000000000472, 0.003490658503988666988 ) ;
#98606=VERTEX_POINT ( 'NONE', #53360 ) ;
#98607=CARTESIAN_POINT ( 'NONE',  ( -12.09999999999999432, 2.500000000000000000, 5.122947341949749323 ) ) ;
#98608=AXIS2_PLACEMENT_3D ( 'NONE', #67238, #126852, #35256 ) ;
#98609=CIRCLE ( 'NONE', #52659, 0.1000000000000000472 ) ;
#98610=DIRECTION ( 'NONE',  ( 0.000000000000000000, 1.000000000000000000, 0.000000000000000000 ) ) ;
#98611=FACE_OUTER_BOUND ( 'NONE', #65865, .T. ) ;
#98612=ORIENTED_EDGE ( 'NONE', *, *, #120509, .F. ) ;
#98613=EDGE_CURVE ( 'NONE', #38111, #21644, #120572, .T. ) ;
#98614=AXIS2_PLACEMENT_3D ( 'NONE', #98474, #107003, #57936 ) ;
#98615=ORIENTED_EDGE ( 'NONE', *, *, #70273, .T. ) ;
#98616=CARTESIAN_POINT ( 'NONE',  ( -6.650000000000019007, 12.50000000000000000, -5.802370205355749988 ) ) ;
#98617=AXIS2_PLACEMENT_3D ( 'NONE', #106867, #38826, #78071 ) ;
#98618=ORIENTED_EDGE ( 'NONE', *, *, #42360, .T. ) ;
#98619=ORIENTED_EDGE ( 'NONE', *, *, #26506, .F. ) ;
#98620=AXIS2_PLACEMENT_3D ( 'NONE', #5454, #6723, #95784 ) ;
#98621=EDGE_LOOP ( 'NONE', ( #63809, #27151, #81707, #37541 ) ) ;
#98622=AXIS2_PLACEMENT_3D ( 'NONE', #24021, #103869, #54119 ) ;
#98623=DIRECTION ( 'NONE',  ( 0.000000000000000000, 0.000000000000000000, -1.000000000000000000 ) ) ;
#98624=EDGE_CURVE ( 'NONE', #30477, #106999, #24432, .T. ) ;
#98625=AXIS2_PLACEMENT_3D ( 'NONE', #26554, #66466, #56629 ) ;
#98626=CARTESIAN_POINT ( 'NONE',  ( -5.000000000000022204, 2.500000000000000000, -0.5928203230275541635 ) ) ;
#98627=DIRECTION ( 'NONE',  ( 0.000000000000000000, -0.9999939076577903929, 0.003490651415223739937 ) ) ;
#98628=ADVANCED_FACE ( 'NONE', ( #113557 ), #33708, .T. ) ;
#98629=CARTESIAN_POINT ( 'NONE',  ( 9.999999999999911182, 2.500000000000000000, 5.022947341949748790 ) ) ;
#98630=ORIENTED_EDGE ( 'NONE', *, *, #121060, .T. ) ;
#98631=EDGE_CURVE ( 'NONE', #77225, #27, #93277, .T. ) ;
#98632=CIRCLE ( 'NONE', #121631, 0.06509327318403745899 ) ;
#98633=DIRECTION ( 'NONE',  ( 0.000000000000000000, 0.000000000000000000, 1.000000000000000000 ) ) ;
#98634=ORIENTED_EDGE ( 'NONE', *, *, #91687, .F. ) ;
#98635=DIRECTION ( 'NONE',  ( -0.000000000000000000, 1.000000000000000000, -0.000000000000000000 ) ) ;
#98636=CARTESIAN_POINT ( 'NONE',  ( 18.20334136263913294, -2.532871263996626432, -4.817802756305527900 ) ) ;
#98637=CARTESIAN_POINT ( 'NONE',  ( 18.09676523922516367, 2.526776815559057532, 2.684906793684505022 ) ) ;
#98638=DIRECTION ( 'NONE',  ( -0.000000000000000000, 1.000000000000000000, -0.000000000000000000 ) ) ;
#98639=ADVANCED_FACE ( 'NONE', ( #103092 ), #32456, .T. ) ;
#98640=DIRECTION ( 'NONE',  ( 0.000000000000000000, 0.000000000000000000, 1.000000000000000000 ) ) ;
#98641=EDGE_CURVE ( 'NONE', #125586, #45052, #11493, .T. ) ;
#98642=EDGE_LOOP ( 'NONE', ( #28357, #129222 ) ) ;
#98643=EDGE_CURVE ( 'NONE', #10889, #126164, #108139, .T. ) ;
#98644=EDGE_CURVE ( 'NONE', #8444, #79920, #129105, .T. ) ;
#98645=ORIENTED_EDGE ( 'NONE', *, *, #125952, .F. ) ;
#98646=ORIENTED_EDGE ( 'NONE', *, *, #40992, .T. ) ;
#98647=ORIENTED_EDGE ( 'NONE', *, *, #72240, .F. ) ;
#98648=ORIENTED_EDGE ( 'NONE', *, *, #19400, .F. ) ;
#98649=DIRECTION ( 'NONE',  ( 0.000000000000000000, 1.000000000000000000, 0.000000000000000000 ) ) ;
#98650=CARTESIAN_POINT ( 'NONE',  ( 1.249999999999953815, 2.500000000000000000, -2.857883832488653741 ) ) ;
#98651=CARTESIAN_POINT ( 'NONE',  ( -13.54999999999998828, 2.500000000000000000, -2.511473670974875727 ) ) ;
#98652=FACE_BOUND ( 'NONE', #109833, .T. ) ;
#98653=CARTESIAN_POINT ( 'NONE',  ( -11.89999999999999680, 12.50000000000000000, -4.741630453620013341 ) ) ;
#98654=DIRECTION ( 'NONE',  ( 0.000000000000000000, 0.000000000000000000, -1.000000000000000000 ) ) ;
#98655=EDGE_CURVE ( 'NONE', #11709, #58497, #42917, .T. ) ;
#98656=DIRECTION ( 'NONE',  ( 0.000000000000000000, 1.000000000000000000, 0.000000000000000000 ) ) ;
#98657=DIRECTION ( 'NONE',  ( 0.000000000000000000, 1.000000000000000000, 0.000000000000000000 ) ) ;
#98658=AXIS2_PLACEMENT_3D ( 'NONE', #31875, #39145, #8993 ) ;
#98659=VECTOR ( 'NONE', #78620, 1000.000000000000000 ) ;
#98661=AXIS2_PLACEMENT_3D ( 'NONE', #110039, #61596, #10527 ) ;
#98662=CARTESIAN_POINT ( 'NONE',  ( -1.450000000000035039, 12.50000000000000000, -2.446380397790840266 ) ) ;
#98663=LINE ( 'NONE', #79057, #70029 ) ;
#98664=AXIS2_PLACEMENT_3D ( 'NONE', #103663, #2881, #32997 ) ;
#98665=CIRCLE ( 'NONE', #40202, 0.06509327318403745899 ) ;
#98666=DIRECTION ( 'NONE',  ( -0.000000000000000000, 1.000000000000000000, -0.000000000000000000 ) ) ;
#98667=AXIS2_PLACEMENT_3D ( 'NONE', #91972, #121421, #50134 ) ;
#98668=VERTEX_POINT ( 'NONE', #92630 ) ;
#98669=ORIENTED_EDGE ( 'NONE', *, *, #81028, .T. ) ;
#98670=ORIENTED_EDGE ( 'NONE', *, *, #113076, .T. ) ;
#98671=ORIENTED_EDGE ( 'NONE', *, *, #3738, .F. ) ;
#98672=CIRCLE ( 'NONE', #52716, 0.09999999999999982514 ) ;
#98673=LINE ( 'NONE', #78432, #117023 ) ;
#98674=CIRCLE ( 'NONE', #77739, 0.06509327318403745899 ) ;
#98675=DIRECTION ( 'NONE',  ( -0.000000000000000000, 1.000000000000000000, -0.000000000000000000 ) ) ;
#98676=FACE_BOUND ( 'NONE', #82194, .T. ) ;
#98677=CARTESIAN_POINT ( 'NONE',  ( 11.24999999999994316, 2.500000000000000000, 2.165063509461097713 ) ) ;
#98678=ORIENTED_EDGE ( 'NONE', *, *, #17928, .T. ) ;
#98679=CARTESIAN_POINT ( 'NONE',  ( 4.399999999999940847, 2.500000000000000000, -4.676537180435977881 ) ) ;
#98680=DIRECTION ( 'NONE',  ( -0.000000000000000000, 1.000000000000000000, -0.000000000000000000 ) ) ;
#98681=DIRECTION ( 'NONE',  ( 0.000000000000000000, 0.000000000000000000, 1.000000000000000000 ) ) ;
#98682=DIRECTION ( 'NONE',  ( -0.000000000000000000, 1.000000000000000000, -0.000000000000000000 ) ) ;
#98683=VERTEX_POINT ( 'NONE', #72360 ) ;
#98685=ADVANCED_FACE ( 'NONE', ( #2297 ), #30802, .T. ) ;
#98686=ORIENTED_EDGE ( 'NONE', *, *, #27946, .F. ) ;
#98687=EDGE_LOOP ( 'NONE', ( #104457, #84426 ) ) ;
#98688=CARTESIAN_POINT ( 'NONE',  ( -8.749999999999976907, 12.50000000000000000, -6.495190528383297135 ) ) ;
#98689=CARTESIAN_POINT ( 'NONE',  ( -3.350000000000028511, 12.50000000000000000, -1.472243186433550122 ) ) ;
#98690=EDGE_LOOP ( 'NONE', ( #824, #22762 ) ) ;
#98691=AXIS2_PLACEMENT_3D ( 'NONE', #80288, #91381, #48903 ) ;
#98692=CARTESIAN_POINT ( 'NONE',  ( 3.749999999999942268, 2.500000000000000000, -5.702370205355749455 ) ) ;
#98693=CARTESIAN_POINT ( 'NONE',  ( -2.100000000000033840, 2.500000000000000000, 5.022947341949748790 ) ) ;
#98694=ORIENTED_EDGE ( 'NONE', *, *, #79850, .F. ) ;
#98695=DIRECTION ( 'NONE',  ( 0.000000000000000000, 1.000000000000000000, 0.000000000000000000 ) ) ;
#98696=ORIENTED_EDGE ( 'NONE', *, *, #33768, .F. ) ;
#98697=ADVANCED_FACE ( 'NONE', ( #122735 ), #101887, .T. ) ;
#98698=DIRECTION ( 'NONE',  ( -0.000000000000000000, -1.000000000000000000, -0.000000000000000000 ) ) ;
#98699=CONICAL_SURFACE ( 'NONE', #94504, 0.1000000000000002554, 0.003490658503988666988 ) ;
#98700=ORIENTED_EDGE ( 'NONE', *, *, #100692, .F. ) ;
#98701=CARTESIAN_POINT ( 'NONE',  ( 1.449999999999952216, 12.50000000000000000, -2.446380397790840266 ) ) ;
#98702=AXIS2_PLACEMENT_3D ( 'NONE', #126611, #7455, #88610 ) ;
#98703=FACE_BOUND ( 'NONE', #59777, .T. ) ;
#98704=AXIS2_PLACEMENT_3D ( 'NONE', #42113, #92489, #33589 ) ;
#98705=VERTEX_POINT ( 'NONE', #36307 ) ;
#98706=CIRCLE ( 'NONE', #84044, 0.06509327318403743123 ) ;
#98708=EDGE_LOOP ( 'NONE', ( #52486, #106932 ) ) ;
#98709=CARTESIAN_POINT ( 'NONE',  ( -3.350000000000028511, 2.500000000000000000, -2.957883832488653830 ) ) ;
#98710=FACE_OUTER_BOUND ( 'NONE', #114041, .T. ) ;
#98711=DIRECTION ( 'NONE',  ( -0.000000000000000000, -1.000000000000000000, -0.000000000000000000 ) ) ;
#98712=CARTESIAN_POINT ( 'NONE',  ( -7.499999999999980460, 2.500000000000000000, -4.330127018922201643 ) ) ;
#98713=DIRECTION ( 'NONE',  ( 0.000000000000000000, -0.000000000000000000, 1.000000000000000000 ) ) ;
#98714=VECTOR ( 'NONE', #97206, 1000.000000000000000 ) ;
#98715=ORIENTED_EDGE ( 'NONE', *, *, #4292, .T. ) ;
#98716=ORIENTED_EDGE ( 'NONE', *, *, #104221, .T. ) ;
#98717=CIRCLE ( 'NONE', #40164, 0.06509327318403745899 ) ;
#98718=ORIENTED_EDGE ( 'NONE', *, *, #111179, .F. ) ;
#98719=DIRECTION ( 'NONE',  ( 0.000000000000000000, 0.000000000000000000, 1.000000000000000000 ) ) ;
#98720=CARTESIAN_POINT ( 'NONE',  ( 2.099999999999948574, 2.500000000000000000, 4.330127018922196314 ) ) ;
#98721=AXIS2_PLACEMENT_3D ( 'NONE', #95537, #66060, #25483 ) ;
#98722=CIRCLE ( 'NONE', #90403, 0.09999999999999982514 ) ;
#98723=CIRCLE ( 'NONE', #25557, 0.1000000000000002554 ) ;
#98724=CARTESIAN_POINT ( 'NONE',  ( 12.89999999999990266, 2.500000000000000000, -3.737306695894649700 ) ) ;
#98725=VERTEX_POINT ( 'NONE', #34373 ) ;
#98726=VERTEX_POINT ( 'NONE', #15335 ) ;
#98727=EDGE_LOOP ( 'NONE', ( #11722, #112279, #82884, #12432 ) ) ;
#98728=CARTESIAN_POINT ( 'NONE',  ( 1.649999999999951061, 12.50000000000000000, -6.495190528383302464 ) ) ;
#98729=AXIS2_PLACEMENT_3D ( 'NONE', #56963, #6549, #66788 ) ;
#98730=FACE_OUTER_BOUND ( 'NONE', #45917, .T. ) ;
#98731=EDGE_CURVE ( 'NONE', #4941, #32170, #125940, .T. ) ;
#98733=DIRECTION ( 'NONE',  ( 0.000000000000000000, 0.000000000000000000, 1.000000000000000000 ) ) ;
#98734=DIRECTION ( 'NONE',  ( -0.000000000000000000, 1.000000000000000000, -0.000000000000000000 ) ) ;
#98735=DIRECTION ( 'NONE',  ( -0.000000000000000000, -1.000000000000000000, -0.000000000000000000 ) ) ;
#98737=DIRECTION ( 'NONE',  ( -4.274815082592931898E-19, -0.9999939076577903929, -0.003490651415223739937 ) ) ;
#98738=DIRECTION ( 'NONE',  ( 0.000000000000000000, 0.000000000000000000, -1.000000000000000000 ) ) ;
#98739=EDGE_CURVE ( 'NONE', #59330, #103763, #54623, .T. ) ;
#98740=VERTEX_POINT ( 'NONE', #105009 ) ;
#98741=ORIENTED_EDGE ( 'NONE', *, *, #6656, .F. ) ;
#98742=FACE_OUTER_BOUND ( 'NONE', #92700, .T. ) ;
#98744=EDGE_CURVE ( 'NONE', #81857, #26026, #78922, .T. ) ;
#98745=ORIENTED_EDGE ( 'NONE', *, *, #121797, .T. ) ;
#98746=EDGE_CURVE ( 'NONE', #81852, #51338, #37057, .T. ) ;
#98747=VERTEX_POINT ( 'NONE', #36941 ) ;
#98748=ADVANCED_FACE ( 'NONE', ( #26474 ), #24526, .T. ) ;
#98750=CARTESIAN_POINT ( 'NONE',  ( 3.349999999999943689, 12.50000000000000000, 2.099970236277060032 ) ) ;
#98752=DIRECTION ( 'NONE',  ( -0.000000000000000000, 1.000000000000000000, -0.000000000000000000 ) ) ;
#98753=LINE ( 'NONE', #9093, #52721 ) ;
#98754=DIRECTION ( 'NONE',  ( -0.000000000000000000, 1.000000000000000000, -0.000000000000000000 ) ) ;
#98755=VECTOR ( 'NONE', #89352, 1000.000000000000000 ) ;
#98756=CARTESIAN_POINT ( 'NONE',  ( 6.049999999999934097, 2.500000000000000000, 6.048780366869521252 ) ) ;
#98757=CARTESIAN_POINT ( 'NONE',  ( -4.400000000000028777, 2.500000000000000000, -4.083716857408426826 ) ) ;
#98758=AXIS2_PLACEMENT_3D ( 'NONE', #101466, #64107, #63474 ) ;
#98759=CIRCLE ( 'NONE', #92504, 0.06509327318403745899 ) ;
#98760=ADVANCED_FACE ( 'NONE', ( #6789 ), #24535, .T. ) ;
#98761=PLANE ( 'NONE',  #102286 ) ;
#98762=ADVANCED_FACE ( 'NONE', ( #15981 ), #85151, .T. ) ;
#98763=CIRCLE ( 'NONE', #42346, 0.06509327318403743123 ) ;
#98764=ADVANCED_FACE ( 'NONE', ( #44831 ), #62193, .T. ) ;
#98765=VERTEX_POINT ( 'NONE', #126613 ) ;
#98766=VECTOR ( 'NONE', #68677, 1000.000000000000000 ) ;
#98767=AXIS2_PLACEMENT_3D ( 'NONE', #104681, #105346, #6456 ) ;
#98768=EDGE_LOOP ( 'NONE', ( #70101, #58030 ) ) ;
#98770=CIRCLE ( 'NONE', #48611, 0.06509327318403743123 ) ;
#98772=EDGE_LOOP ( 'NONE', ( #87962, #67881, #65496, #19472 ) ) ;
#98773=ORIENTED_EDGE ( 'NONE', *, *, #104424, .T. ) ;
#98774=FACE_OUTER_BOUND ( 'NONE', #108271, .T. ) ;
#98775=DIRECTION ( 'NONE',  ( 0.000000000000000000, -0.000000000000000000, 1.000000000000000000 ) ) ;
#98776=CONICAL_SURFACE ( 'NONE', #38254, 0.1000000000000002554, 0.003490658503988666988 ) ;
#98777=VERTEX_POINT ( 'NONE', #94550 ) ;
#98778=CARTESIAN_POINT ( 'NONE',  ( -7.300000000000016698, 2.500000000000000000, -0.2464101615137783419 ) ) ;
#98779=DIRECTION ( 'NONE',  ( 0.000000000000000000, -0.9999939076577903929, 0.003490651415223739937 ) ) ;
#98780=DIRECTION ( 'NONE',  ( -0.000000000000000000, 1.000000000000000000, -0.000000000000000000 ) ) ;
#98781=DIRECTION ( 'NONE',  ( 0.000000000000000000, 1.000000000000000000, 0.000000000000000000 ) ) ;
#98782=EDGE_LOOP ( 'NONE', ( #83442, #129017 ) ) ;
#98783=DIRECTION ( 'NONE',  ( -0.000000000000000000, -1.000000000000000000, -0.000000000000000000 ) ) ;
#98784=DIRECTION ( 'NONE',  ( -0.000000000000000000, -1.000000000000000000, -0.000000000000000000 ) ) ;
#98785=ORIENTED_EDGE ( 'NONE', *, *, #89517, .F. ) ;
#98786=VERTEX_POINT ( 'NONE', #76221 ) ;
#98787=EDGE_LOOP ( 'NONE', ( #50169, #15806, #118668, #66029 ) ) ;
#98788=ORIENTED_EDGE ( 'NONE', *, *, #93266, .F. ) ;
#98789=CARTESIAN_POINT ( 'NONE',  ( -3.749999999999991118, 12.50000000000000000, -2.099970236277064473 ) ) ;
#98790=AXIS2_PLACEMENT_3D ( 'NONE', #6838, #118107, #76902 ) ;
#98791=CARTESIAN_POINT ( 'NONE',  ( 5.399999999999934630, 2.500000000000000000, 0.7928203230275495672 ) ) ;
#98792=AXIS2_PLACEMENT_3D ( 'NONE', #128663, #17362, #38997 ) ;
#98793=VECTOR ( 'NONE', #66173, 1000.000000000000000 ) ;
#98794=VERTEX_POINT ( 'NONE', #14687 ) ;
#98795=CARTESIAN_POINT ( 'NONE',  ( -9.550000000000007816, 2.500000000000000000, -6.595190528383296780 ) ) ;
#98796=FACE_OUTER_BOUND ( 'NONE', #128307, .T. ) ;
#98797=CARTESIAN_POINT ( 'NONE',  ( 1.649999999999951505, 12.50000000000000000, 2.922977105672686982 ) ) ;
#98798=LINE ( 'NONE', #47785, #81795 ) ;
#98799=ADVANCED_FACE ( 'NONE', ( #124675 ), #126938, .T. ) ;
#98800=AXIS2_PLACEMENT_3D ( 'NONE', #54685, #59894, #129279 ) ;
#98801=AXIS2_PLACEMENT_3D ( 'NONE', #71890, #93448, #33264 ) ;
#98802=EDGE_CURVE ( 'NONE', #40796, #10550, #22494, .T. ) ;
#98803=VECTOR ( 'NONE', #29021, 1000.000000000000000 ) ;
#98804=VERTEX_POINT ( 'NONE', #25168 ) ;
#98805=LINE ( 'NONE', #9145, #41620 ) ;
#98806=AXIS2_PLACEMENT_3D ( 'NONE', #42130, #4752, #82714 ) ;
#98807=EDGE_CURVE ( 'NONE', #120378, #896, #20322, .T. ) ;
#98808=ORIENTED_EDGE ( 'NONE', *, *, #122057, .T. ) ;
#98809=ORIENTED_EDGE ( 'NONE', *, *, #25524, .T. ) ;
#98810=DIRECTION ( 'NONE',  ( 0.000000000000000000, 0.000000000000000000, -1.000000000000000000 ) ) ;
#98811=CARTESIAN_POINT ( 'NONE',  ( 3.349999999999941025, 2.500000000000000000, 7.188010851410848723 ) ) ;
#98812=FACE_BOUND ( 'NONE', #105179, .T. ) ;
#98813=DIRECTION ( 'NONE',  ( 0.000000000000000000, 1.000000000000000000, 0.000000000000000000 ) ) ;
#98814=CARTESIAN_POINT ( 'NONE',  ( -1.850000000000033840, 2.500000000000000000, 6.841600689897072485 ) ) ;
#98815=AXIS2_PLACEMENT_3D ( 'NONE', #98814, #30108, #70020 ) ;
#98816=EDGE_CURVE ( 'NONE', #71034, #91607, #124877, .T. ) ;
#98817=CIRCLE ( 'NONE', #25660, 0.06509327318403745899 ) ;
#98819=AXIS2_PLACEMENT_3D ( 'NONE', #119050, #59513, #99423 ) ;
#98820=AXIS2_PLACEMENT_3D ( 'NONE', #72657, #41274, #53013 ) ;
#98821=VERTEX_POINT ( 'NONE', #45482 ) ;
#98822=DIRECTION ( 'NONE',  ( 0.000000000000000000, -0.000000000000000000, 1.000000000000000000 ) ) ;
#98823=CARTESIAN_POINT ( 'NONE',  ( -9.800000000000006040, 12.50000000000000000, 4.676537180435972552 ) ) ;
#98824=CARTESIAN_POINT ( 'NONE',  ( 6.649999999999931077, 2.500000000000000000, -6.395190528383301931 ) ) ;
#98825=DIRECTION ( 'NONE',  ( 0.000000000000000000, 0.000000000000000000, -1.000000000000000000 ) ) ;
#98826=EDGE_LOOP ( 'NONE', ( #127842, #29501 ) ) ;
#98827=DIRECTION ( 'NONE',  ( -0.000000000000000000, 1.000000000000000000, -0.000000000000000000 ) ) ;
#98828=DIRECTION ( 'NONE',  ( 0.000000000000000000, 0.000000000000000000, 1.000000000000000000 ) ) ;
#98829=VERTEX_POINT ( 'NONE', #103744 ) ;
#98830=ORIENTED_EDGE ( 'NONE', *, *, #19491, .T. ) ;
#98831=CARTESIAN_POINT ( 'NONE',  ( 6.899999999999926636, 2.500000000000000000, 0.3464101615137736845 ) ) ;
#98832=DIRECTION ( 'NONE',  ( 0.000000000000000000, 0.000000000000000000, 1.000000000000000000 ) ) ;
#98833=EDGE_CURVE ( 'NONE', #112209, #36772, #27114, .T. ) ;
#98834=FACE_BOUND ( 'NONE', #88842, .T. ) ;
#98835=CARTESIAN_POINT ( 'NONE',  ( 9.599999999999914380, 2.500000000000000000, -4.230127018922201998 ) ) ;
#98837=CARTESIAN_POINT ( 'NONE',  ( 10.64999999999990976, 2.500000000000000000, -6.841600689897077814 ) ) ;
#98838=CIRCLE ( 'NONE', #90530, 0.06509327318403745899 ) ;
#98839=ORIENTED_EDGE ( 'NONE', *, *, #87402, .F. ) ;
#98840=CARTESIAN_POINT ( 'NONE',  ( 7.899999999999924860, 2.500000000000000000, -5.122947341949753763 ) ) ;
#98841=CIRCLE ( 'NONE', #103050, 0.09999999999999982514 ) ;
#98843=ORIENTED_EDGE ( 'NONE', *, *, #2018, .T. ) ;
#98844=DIRECTION ( 'NONE',  ( 0.000000000000000000, -0.9999939076577903929, 0.003490651415223739937 ) ) ;
#98845=DIRECTION ( 'NONE',  ( -4.274815082592931898E-19, -0.9999939076577903929, -0.003490651415223739937 ) ) ;
#98846=AXIS2_PLACEMENT_3D ( 'NONE', #88152, #128110, #106525 ) ;
#98847=EDGE_CURVE ( 'NONE', #76584, #103548, #9855, .T. ) ;
#98848=AXIS2_PLACEMENT_3D ( 'NONE', #121577, #22769, #41120 ) ;
#98849=AXIS2_PLACEMENT_3D ( 'NONE', #14712, #35043, #54642 ) ;
#98850=FACE_OUTER_BOUND ( 'NONE', #40624, .T. ) ;
#98851=DIRECTION ( 'NONE',  ( 0.000000000000000000, 0.000000000000000000, 1.000000000000000000 ) ) ;
#98852=AXIS2_PLACEMENT_3D ( 'NONE', #21035, #83195, #62268 ) ;
#98853=CIRCLE ( 'NONE', #4856, 0.06509327318403745899 ) ;
#98854=ORIENTED_EDGE ( 'NONE', *, *, #114715, .F. ) ;
#98855=VECTOR ( 'NONE', #25862, 1000.000000000000000 ) ;
#98856=DIRECTION ( 'NONE',  ( 0.000000000000000000, 0.000000000000000000, 1.000000000000000000 ) ) ;
#98857=FACE_OUTER_BOUND ( 'NONE', #26134, .T. ) ;
#98858=DIRECTION ( 'NONE',  ( 0.000000000000000000, -0.9999939076577903929, 0.003490651415223739937 ) ) ;
#98859=AXIS2_PLACEMENT_3D ( 'NONE', #56058, #114976, #96003 ) ;
#98860=DIRECTION ( 'NONE',  ( -4.274815082592931898E-19, -0.9999939076577903929, -0.003490651415223739937 ) ) ;
#98861=CIRCLE ( 'NONE', #82156, 0.06509327318403745899 ) ;
#98863=ORIENTED_EDGE ( 'NONE', *, *, #91246, .T. ) ;
#98864=EDGE_CURVE ( 'NONE', #113013, #24462, #119351, .T. ) ;
#98865=CARTESIAN_POINT ( 'NONE',  ( 16.56576425165006938, 1.499999999999999112, 6.084390597445819004 ) ) ;
#98866=CIRCLE ( 'NONE', #80106, 0.06509327318403741736 ) ;
#98867=ORIENTED_EDGE ( 'NONE', *, *, #119490, .F. ) ;
#98868=FACE_OUTER_BOUND ( 'NONE', #1680, .T. ) ;
#98870=CARTESIAN_POINT ( 'NONE',  ( -6.250000000000015987, 12.50000000000000000, 1.472243186433545459 ) ) ;
#98871=DIRECTION ( 'NONE',  ( 0.000000000000000000, 0.000000000000000000, -1.000000000000000000 ) ) ;
#98872=ORIENTED_EDGE ( 'NONE', *, *, #104454, .T. ) ;
#98873=DIRECTION ( 'NONE',  ( 0.000000000000000000, 0.000000000000000000, 1.000000000000000000 ) ) ;
#98874=CARTESIAN_POINT ( 'NONE',  ( -12.89999999999999325, 2.500000000000000000, -3.737306695894647035 ) ) ;
#98875=LINE ( 'NONE', #20328, #98659 ) ;
#98876=EDGE_CURVE ( 'NONE', #73152, #97131, #51720, .T. ) ;
#98878=DIRECTION ( 'NONE',  ( 0.000000000000000000, 0.000000000000000000, 1.000000000000000000 ) ) ;
#98879=DIRECTION ( 'NONE',  ( 0.000000000000000000, 0.000000000000000000, -1.000000000000000000 ) ) ;
#98880=CONICAL_SURFACE ( 'NONE', #126064, 0.1000000000000002554, 0.003490658503988666988 ) ;
#98881=ORIENTED_EDGE ( 'NONE', *, *, #92835, .F. ) ;
#98882=ORIENTED_EDGE ( 'NONE', *, *, #57527, .T. ) ;
#98883=CARTESIAN_POINT ( 'NONE',  ( 4.399999999999937295, 12.50000000000000000, 3.983716857408420964 ) ) ;
#98884=ORIENTED_EDGE ( 'NONE', *, *, #96476, .T. ) ;
#98885=CARTESIAN_POINT ( 'NONE',  ( -4.600000000000024514, 2.500000000000000000, 4.922947341949748257 ) ) ;
#98886=ORIENTED_EDGE ( 'NONE', *, *, #80240, .F. ) ;
#98887=ORIENTED_EDGE ( 'NONE', *, *, #78435, .F. ) ;
#98888=VERTEX_POINT ( 'NONE', #68967 ) ;
#98889=CARTESIAN_POINT ( 'NONE',  ( 17.50000000000000000, -1.666666666666663632, -3.999999999999997335 ) ) ;
#98890=CIRCLE ( 'NONE', #19467, 0.1000000000000002554 ) ;
#98891=CIRCLE ( 'NONE', #689, 0.06509327318403745899 ) ;
#98892=DIRECTION ( 'NONE',  ( 0.000000000000000000, 0.000000000000000000, -1.000000000000000000 ) ) ;
#98893=AXIS2_PLACEMENT_3D ( 'NONE', #49144, #47196, #30144 ) ;
#98894=DIRECTION ( 'NONE',  ( -0.000000000000000000, 1.000000000000000000, -0.000000000000000000 ) ) ;
#98895=EDGE_CURVE ( 'NONE', #55057, #40266, #47517, .T. ) ;
#98897=CARTESIAN_POINT ( 'NONE',  ( 5.849999999999931255, 2.500000000000000000, 2.957883832488649389 ) ) ;
#98898=LINE ( 'NONE', #94234, #113406 ) ;
#98899=LINE ( 'NONE', #39369, #114525 ) ;
#98900=DIRECTION ( 'NONE',  ( 0.000000000000000000, 0.000000000000000000, 1.000000000000000000 ) ) ;
#98901=AXIS2_PLACEMENT_3D ( 'NONE', #106704, #56316, #126361 ) ;
#98902=AXIS2_PLACEMENT_3D ( 'NONE', #6323, #84260, #24069 ) ;
#98903=DIRECTION ( 'NONE',  ( -4.274815082592931898E-19, -0.9999939076577903929, -0.003490651415223739937 ) ) ;
#98904=EDGE_LOOP ( 'NONE', ( #23309, #4238, #48703, #126842 ) ) ;
#98905=CIRCLE ( 'NONE', #128161, 0.06509327318403745899 ) ;
#98906=ADVANCED_FACE ( 'NONE', ( #59831 ), #68318, .T. ) ;
#98907=VERTEX_POINT ( 'NONE', #87308 ) ;
#98908=AXIS2_PLACEMENT_3D ( 'NONE', #35543, #66906, #27004 ) ;
#98909=CARTESIAN_POINT ( 'NONE',  ( -8.150000000000012790, 2.500000000000000000, -1.818653347947326138 ) ) ;
#98910=EDGE_CURVE ( 'NONE', #125538, #80531, #3593, .T. ) ;
#98911=ORIENTED_EDGE ( 'NONE', *, *, #78420, .T. ) ;
#98912=ADVANCED_FACE ( 'NONE', ( #10055 ), #66286, .T. ) ;
#98913=EDGE_LOOP ( 'NONE', ( #21299, #78218, #72967, #32021 ) ) ;
#98914=EDGE_CURVE ( 'NONE', #21836, #3798, #93487, .T. ) ;
#98915=CARTESIAN_POINT ( 'NONE',  ( 5.799999999999931433, 2.500000000000000000, 4.330127018922196314 ) ) ;
#98916=EDGE_CURVE ( 'NONE', #73210, #4103, #18583, .T. ) ;
#98917=CONICAL_SURFACE ( 'NONE', #42501, 0.1000000000000002554, 0.003490658503988666988 ) ;
#98918=CARTESIAN_POINT ( 'NONE',  ( -5.600000000000023626, 2.500000000000000000, -4.776537180435977525 ) ) ;
#98919=DIRECTION ( 'NONE',  ( -0.000000000000000000, 1.000000000000000000, -0.000000000000000000 ) ) ;
#98920=CIRCLE ( 'NONE', #46691, 0.06509327318403745899 ) ;
#98921=CARTESIAN_POINT ( 'NONE',  ( 4.149999999999941735, 12.50000000000000000, -7.253104124594891289 ) ) ;
#98922=AXIS2_PLACEMENT_3D ( 'NONE', #65097, #106335, #125962 ) ;
#98923=CONICAL_SURFACE ( 'NONE', #55000, 0.1000000000000002554, 0.003490658503988666988 ) ;
#98924=EDGE_CURVE ( 'NONE', #107468, #62993, #80961, .T. ) ;
#98925=DIRECTION ( 'NONE',  ( 0.000000000000000000, 0.000000000000000000, 1.000000000000000000 ) ) ;
#98926=ORIENTED_EDGE ( 'NONE', *, *, #3150, .F. ) ;
#98927=EDGE_CURVE ( 'NONE', #34370, #29668, #114398, .T. ) ;
#98928=CONICAL_SURFACE ( 'NONE', #11078, 0.09999999999999982514, 0.003490658503988666988 ) ;
#98929=ADVANCED_FACE ( 'NONE', ( #8109 ), #122727, .T. ) ;
#98930=EDGE_CURVE ( 'NONE', #106895, #122432, #59165, .T. ) ;
#98931=VERTEX_POINT ( 'NONE', #19204 ) ;
#98932=CARTESIAN_POINT ( 'NONE',  ( -12.04999999999999538, 2.500000000000000000, 6.495190528383297135 ) ) ;
#98933=EDGE_CURVE ( 'NONE', #105604, #48799, #28741, .T. ) ;
#98934=VERTEX_POINT ( 'NONE', #78159 ) ;
#98935=AXIS2_PLACEMENT_3D ( 'NONE', #67124, #70874, #16099 ) ;
#98936=LINE ( 'NONE', #9267, #42070 ) ;
#98937=ORIENTED_EDGE ( 'NONE', *, *, #16899, .T. ) ;
#98938=ORIENTED_EDGE ( 'NONE', *, *, #37041, .F. ) ;
#98939=EDGE_CURVE ( 'NONE', #117692, #122978, #79015, .T. ) ;
#98940=DIRECTION ( 'NONE',  ( -4.274815082592931898E-19, -0.9999939076577903929, -0.003490651415223739937 ) ) ;
#98941=LINE ( 'NONE', #68830, #127963 ) ;
#98942=DIRECTION ( 'NONE',  ( 0.000000000000000000, 0.000000000000000000, 1.000000000000000000 ) ) ;
#98943=CARTESIAN_POINT ( 'NONE',  ( 0.1999999999999571565, 2.500000000000000000, 4.083716857408420609 ) ) ;
#98944=CARTESIAN_POINT ( 'NONE',  ( 4.999999999999971578, 2.500000000000000000, -0.1000000000000022815 ) ) ;
#98945=EDGE_LOOP ( 'NONE', ( #51623, #9681 ) ) ;
#98946=CARTESIAN_POINT ( 'NONE',  ( -8.550000000000013145, 12.50000000000000000, -6.906693963081110610 ) ) ;
#98947=CARTESIAN_POINT ( 'NONE',  ( 11.64999999999990443, 2.500000000000000000, -7.188010851410854052 ) ) ;
#98948=AXIS2_PLACEMENT_3D ( 'NONE', #122383, #10472, #123023 ) ;
#98949=CARTESIAN_POINT ( 'NONE',  ( 13.14999999999990088, 12.50000000000000000, 2.446380397790835826 ) ) ;
#98950=CARTESIAN_POINT ( 'NONE',  ( -11.64999999999999680, 12.50000000000000000, 1.407149913249508000 ) ) ;
#98951=CARTESIAN_POINT ( 'NONE',  ( -1.250000000000037970, 2.500000000000000000, 2.957883832488649389 ) ) ;
#98952=ORIENTED_EDGE ( 'NONE', *, *, #89888, .T. ) ;
#98953=AXIS2_PLACEMENT_3D ( 'NONE', #42311, #82233, #50838 ) ;
#98954=VERTEX_POINT ( 'NONE', #50001 ) ;
#98955=AXIS2_PLACEMENT_3D ( 'NONE', #114341, #34521, #124163 ) ;
#98956=CARTESIAN_POINT ( 'NONE',  ( -2.900000000000029221, 12.50000000000000000, -0.06509327318403970719 ) ) ;
#98957=EDGE_LOOP ( 'NONE', ( #64243, #104555, #7836, #32217 ) ) ;
#98958=CARTESIAN_POINT ( 'NONE',  ( 6.649999999999929301, 2.500000000000000000, 6.395190528383296602 ) ) ;
#98959=CARTESIAN_POINT ( 'NONE',  ( -3.150000000000032330, 2.500000000000000000, -6.248780366869526759 ) ) ;
#98960=AXIS2_PLACEMENT_3D ( 'NONE', #128547, #11319, #38214 ) ;
#98961=CIRCLE ( 'NONE', #38335, 0.1000000000000000472 ) ;
#98962=VECTOR ( 'NONE', #16122, 1000.000000000000000 ) ;
#98963=CIRCLE ( 'NONE', #661, 0.1000000000000002554 ) ;
#98964=VERTEX_POINT ( 'NONE', #89894 ) ;
#98965=LINE ( 'NONE', #49240, #82881 ) ;
#98966=CARTESIAN_POINT ( 'NONE',  ( -9.800000000000006040, 2.500000000000000000, -4.776537180435973973 ) ) ;
#98967=CARTESIAN_POINT ( 'NONE',  ( -12.49999999999999467, 2.500000000000000000, 0.6928203230275535862 ) ) ;
#98968=DIRECTION ( 'NONE',  ( 0.000000000000000000, -0.000000000000000000, 1.000000000000000000 ) ) ;
#98969=ORIENTED_EDGE ( 'NONE', *, *, #52508, .T. ) ;
#98970=CIRCLE ( 'NONE', #69427, 0.06509327318403745899 ) ;
#98971=EDGE_CURVE ( 'NONE', #93899, #119348, #89457, .T. ) ;
#98972=CARTESIAN_POINT ( 'NONE',  ( 2.899999999999945732, 2.500000000000000000, -0.1000000000000023925 ) ) ;
#98973=EDGE_CURVE ( 'NONE', #25372, #99497, #104037, .T. ) ;
#98974=ORIENTED_EDGE ( 'NONE', *, *, #125597, .F. ) ;
#98975=CARTESIAN_POINT ( 'NONE',  ( -4.350000000000027178, 2.500000000000000000, -6.741600689897077281 ) ) ;
#98976=LINE ( 'NONE', #30260, #97853 ) ;
#98977=DIRECTION ( 'NONE',  ( 0.000000000000000000, 0.000000000000000000, -1.000000000000000000 ) ) ;
#98978=VECTOR ( 'NONE', #70175, 1000.000000000000000 ) ;
#98979=EDGE_CURVE ( 'NONE', #35537, #83674, #43423, .T. ) ;
#98980=ORIENTED_EDGE ( 'NONE', *, *, #34484, .F. ) ;
#98981=CARTESIAN_POINT ( 'NONE',  ( 5.849999999999932143, 2.500000000000000000, 2.165063509461097713 ) ) ;
#98982=VERTEX_POINT ( 'NONE', #48694 ) ;
#98983=CARTESIAN_POINT ( 'NONE',  ( 5.649999999999936406, 12.50000000000000000, -6.841600689897077814 ) ) ;
#98984=DIRECTION ( 'NONE',  ( 0.000000000000000000, 0.000000000000000000, 1.000000000000000000 ) ) ;
#98985=DIRECTION ( 'NONE',  ( -0.000000000000000000, -1.000000000000000000, -0.000000000000000000 ) ) ;
#98986=CONICAL_SURFACE ( 'NONE', #86364, 0.09999999999999999167, 0.003490658503988666988 ) ;
#98987=ORIENTED_EDGE ( 'NONE', *, *, #15566, .T. ) ;
#98988=AXIS2_PLACEMENT_3D ( 'NONE', #38162, #78753, #76802 ) ;
#98989=AXIS2_PLACEMENT_3D ( 'NONE', #23304, #22694, #21380 ) ;
#98990=CARTESIAN_POINT ( 'NONE',  ( -0.8500000000000386136, 12.50000000000000000, 2.857883832488649301 ) ) ;
#98991=CARTESIAN_POINT ( 'NONE',  ( -11.84999999999999787, 2.500000000000000000, -6.741600689897073728 ) ) ;
#98992=ORIENTED_EDGE ( 'NONE', *, *, #116899, .T. ) ;
#98993=FACE_OUTER_BOUND ( 'NONE', #124027, .T. ) ;
#98994=AXIS2_PLACEMENT_3D ( 'NONE', #83073, #12378, #93525 ) ;
#98995=EDGE_LOOP ( 'NONE', ( #82782, #102005, #86764, #107556 ) ) ;
#98996=CIRCLE ( 'NONE', #111613, 0.1000000000000002554 ) ;
#98997=DIRECTION ( 'NONE',  ( -0.000000000000000000, 1.000000000000000000, -0.000000000000000000 ) ) ;
#98998=AXIS2_PLACEMENT_3D ( 'NONE', #36447, #66514, #127390 ) ;
#98999=ORIENTED_EDGE ( 'NONE', *, *, #65640, .T. ) ;
#99002=ORIENTED_EDGE ( 'NONE', *, *, #1060, .T. ) ;
#99003=ORIENTED_EDGE ( 'NONE', *, *, #57740, .F. ) ;
#99004=CIRCLE ( 'NONE', #73970, 0.09999999999999982514 ) ;
#99005=LINE ( 'NONE', #37522, #76041 ) ;
#99006=DIRECTION ( 'NONE',  ( 0.000000000000000000, 0.000000000000000000, 1.000000000000000000 ) ) ;
#99007=EDGE_LOOP ( 'NONE', ( #74495, #99600 ) ) ;
#99008=DIRECTION ( 'NONE',  ( 0.000000000000000000, 1.000000000000000000, 0.000000000000000000 ) ) ;
#99009=ADVANCED_FACE ( 'NONE', ( #88611 ), #33047, .T. ) ;
#99011=CONICAL_SURFACE ( 'NONE', #44737, 0.09999999999999982514, 0.003490658503988666988 ) ;
#99012=DIRECTION ( 'NONE',  ( -0.000000000000000000, -1.000000000000000000, -0.000000000000000000 ) ) ;
#99013=CIRCLE ( 'NONE', #96950, 0.06509327318403741736 ) ;
#99014=CONICAL_SURFACE ( 'NONE', #92763, 0.09999999999999999167, 0.003490658503988666988 ) ;
#99016=DIRECTION ( 'NONE',  ( 0.000000000000000000, -0.9999939076577903929, 0.003490651415223739937 ) ) ;
#99017=CARTESIAN_POINT ( 'NONE',  ( 8.349999999999919709, 2.500000000000000000, 7.188010851410848723 ) ) ;
#99018=AXIS2_PLACEMENT_3D ( 'NONE', #40270, #8211, #70365 ) ;
#99019=CARTESIAN_POINT ( 'NONE',  ( -5.800000000000022027, 2.500000000000000000, -4.330127018922201643 ) ) ;
#99020=AXIS2_PLACEMENT_3D ( 'NONE', #25103, #65007, #53297 ) ;
#99021=ORIENTED_EDGE ( 'NONE', *, *, #121783, .F. ) ;
#99022=ORIENTED_EDGE ( 'NONE', *, *, #97501, .F. ) ;
#99023=ORIENTED_EDGE ( 'NONE', *, *, #24263, .T. ) ;
#99024=ORIENTED_EDGE ( 'NONE', *, *, #15713, .F. ) ;
#99025=CARTESIAN_POINT ( 'NONE',  ( -10.65000000000000391, 2.500000000000000000, -6.148780366869522673 ) ) ;
#99026=CARTESIAN_POINT ( 'NONE',  ( 87.50000000000001421, 0.000000000000000000, 0.000000000000000000 ) ) ;
#99027=ADVANCED_FACE ( 'NONE', ( #22474 ), #102309, .T. ) ;
#99028=DIRECTION ( 'NONE',  ( 0.000000000000000000, 0.000000000000000000, -1.000000000000000000 ) ) ;
#99029=ORIENTED_EDGE ( 'NONE', *, *, #52108, .T. ) ;
#99030=FACE_BOUND ( 'NONE', #128256, .T. ) ;
#99031=EDGE_LOOP ( 'NONE', ( #29796, #113418 ) ) ;
#99032=ADVANCED_FACE ( 'NONE', ( #42097 ), #47610, .T. ) ;
#99033=DIRECTION ( 'NONE',  ( -4.274815082592931898E-19, -0.9999939076577903929, -0.003490651415223739937 ) ) ;
#99034=DIRECTION ( 'NONE',  ( -0.000000000000000000, -1.000000000000000000, -0.000000000000000000 ) ) ;
#99035=DIRECTION ( 'NONE',  ( 0.000000000000000000, -0.9999939076577903929, 0.003490651415223739937 ) ) ;
#99036=DIRECTION ( 'NONE',  ( 0.000000000000000000, 0.000000000000000000, -1.000000000000000000 ) ) ;
#99037=CARTESIAN_POINT ( 'NONE',  ( 4.149999999999941735, 12.50000000000000000, -5.802370205355749988 ) ) ;
#99038=CARTESIAN_POINT ( 'NONE',  ( 11.04999999999991189, 2.500000000000000000, -2.511473670974877948 ) ) ;
#99039=DIRECTION ( 'NONE',  ( 0.000000000000000000, 1.000000000000000000, 0.000000000000000000 ) ) ;
#99040=DIRECTION ( 'NONE',  ( 0.000000000000000000, 1.000000000000000000, 0.000000000000000000 ) ) ;
#99041=VECTOR ( 'NONE', #96020, 1000.000000000000000 ) ;
#99042=CIRCLE ( 'NONE', #34302, 0.1000000000000000472 ) ;
#99043=EDGE_CURVE ( 'NONE', #98765, #23160, #53866, .T. ) ;
#99044=PLANE ( 'NONE',  #47687 ) ;
#99045=CARTESIAN_POINT ( 'NONE',  ( -4.600000000000028955, 12.50000000000000000, -4.330127018922201643 ) ) ;
#99046=CIRCLE ( 'NONE', #117801, 0.09999999999999982514 ) ;
#99047=ORIENTED_EDGE ( 'NONE', *, *, #52692, .T. ) ;
#99048=ORIENTED_EDGE ( 'NONE', *, *, #90423, .T. ) ;
#99049=ORIENTED_EDGE ( 'NONE', *, *, #94660, .F. ) ;
#99050=AXIS2_PLACEMENT_3D ( 'NONE', #112166, #99770, #100412 ) ;
#99051=ORIENTED_EDGE ( 'NONE', *, *, #101021, .T. ) ;
#99053=DIRECTION ( 'NONE',  ( -4.274815082592931898E-19, -0.9999939076577903929, -0.003490651415223739937 ) ) ;
#99054=AXIS2_PLACEMENT_3D ( 'NONE', #69107, #39045, #108390 ) ;
#99055=CONICAL_SURFACE ( 'NONE', #92799, 0.09999999999999982514, 0.003490658503988666988 ) ;
#99056=DIRECTION ( 'NONE',  ( 0.000000000000000000, 1.000000000000000000, 0.000000000000000000 ) ) ;
#99058=EDGE_LOOP ( 'NONE', ( #102721, #8142 ) ) ;
#99059=EDGE_LOOP ( 'NONE', ( #51626, #24026 ) ) ;
#99060=EDGE_LOOP ( 'NONE', ( #127357, #3802, #121388, #49304 ) ) ;
#99061=CARTESIAN_POINT ( 'NONE',  ( 3.949999999999940670, 12.50000000000000000, 1.818653347947321475 ) ) ;
#99062=AXIS2_PLACEMENT_3D ( 'NONE', #52927, #91561, #62113 ) ;
#99063=VECTOR ( 'NONE', #36644, 1000.000000000000000 ) ;
#99064=DIRECTION ( 'NONE',  ( 0.000000000000000000, 1.000000000000000000, 0.000000000000000000 ) ) ;
#99065=DIRECTION ( 'NONE',  ( -0.000000000000000000, -1.000000000000000000, -0.000000000000000000 ) ) ;
#99066=PLANE ( 'NONE',  #87649 ) ;
#99067=CARTESIAN_POINT ( 'NONE',  ( 4.399999999999939071, 2.500000000000000000, -0.2464101615137782308 ) ) ;
#99068=DIRECTION ( 'NONE',  ( 0.000000000000000000, -0.000000000000000000, 1.000000000000000000 ) ) ;
#99069=CIRCLE ( 'NONE', #73920, 0.09999999999999982514 ) ;
#99070=FACE_OUTER_BOUND ( 'NONE', #3852, .T. ) ;
#99071=ORIENTED_EDGE ( 'NONE', *, *, #37457, .T. ) ;
#99072=DIRECTION ( 'NONE',  ( 0.000000000000000000, 1.000000000000000000, 0.000000000000000000 ) ) ;
#99073=ORIENTED_EDGE ( 'NONE', *, *, #9112, .T. ) ;
#99074=EDGE_CURVE ( 'NONE', #70902, #77506, #20415, .T. ) ;
#99075=EDGE_LOOP ( 'NONE', ( #89067, #1310, #29031 ) ) ;
#99076=ORIENTED_EDGE ( 'NONE', *, *, #16163, .F. ) ;
#99077=CARTESIAN_POINT ( 'NONE',  ( 0.3999999999999568345, 12.50000000000000000, -3.637306695894650055 ) ) ;
#99078=ORIENTED_EDGE ( 'NONE', *, *, #77039, .F. ) ;
#99079=EDGE_CURVE ( 'NONE', #112495, #84287, #5810, .T. ) ;
#99080=VERTEX_POINT ( 'NONE', #23095 ) ;
#99081=EDGE_CURVE ( 'NONE', #9996, #77958, #12088, .T. ) ;
#99082=AXIS2_PLACEMENT_3D ( 'NONE', #58274, #28161, #49105 ) ;
#99083=DIRECTION ( 'NONE',  ( 0.000000000000000000, 1.000000000000000000, 0.000000000000000000 ) ) ;
#99084=CARTESIAN_POINT ( 'NONE',  ( 6.049999999999930544, 12.50000000000000000, 2.511473670974873507 ) ) ;
#99085=DIRECTION ( 'NONE',  ( 0.000000000000000000, 0.000000000000000000, 1.000000000000000000 ) ) ;
#99086=DIRECTION ( 'NONE',  ( 0.000000000000000000, 0.000000000000000000, 1.000000000000000000 ) ) ;
#99087=EDGE_CURVE ( 'NONE', #106434, #59553, #31631, .T. ) ;
#99088=ADVANCED_FACE ( 'NONE', ( #111463 ), #66459, .T. ) ;
#99089=CARTESIAN_POINT ( 'NONE',  ( -12.89999999999999147, 12.50000000000000000, -4.330127018922198978 ) ) ;
#99090=EDGE_CURVE ( 'NONE', #73842, #102428, #50611, .T. ) ;
#99091=ORIENTED_EDGE ( 'NONE', *, *, #37719, .F. ) ;
#99092=CARTESIAN_POINT ( 'NONE',  ( -13.54999999999999005, 12.50000000000000000, -1.818653347947323917 ) ) ;
#99093=CIRCLE ( 'NONE', #82376, 0.09999999999999982514 ) ;
#99094=AXIS2_PLACEMENT_3D ( 'NONE', #17682, #78572, #118464 ) ;
#99095=ORIENTED_EDGE ( 'NONE', *, *, #19721, .T. ) ;
#99096=CARTESIAN_POINT ( 'NONE',  ( -2.700000000000030820, 12.50000000000000000, 0.3464101615137735735 ) ) ;
#99097=ADVANCED_FACE ( 'NONE', ( #120650 ), #53212, .T. ) ;
#99098=ORIENTED_EDGE ( 'NONE', *, *, #33435, .F. ) ;
#99100=DIRECTION ( 'NONE',  ( 0.000000000000000000, 1.000000000000000000, 0.000000000000000000 ) ) ;
#99102=CARTESIAN_POINT ( 'NONE',  ( 9.599999999999914380, 2.500000000000000000, -4.430127018922202176 ) ) ;
#99103=DIRECTION ( 'NONE',  ( -4.274815082592931898E-19, -0.9999939076577903929, -0.003490651415223739937 ) ) ;
#99104=CONICAL_SURFACE ( 'NONE', #42679, 0.09999999999999982514, 0.003490658503988666988 ) ;
#99105=ORIENTED_EDGE ( 'NONE', *, *, #19711, .T. ) ;
#99106=EDGE_CURVE ( 'NONE', #63978, #90160, #7876, .T. ) ;
#99107=AXIS2_PLACEMENT_3D ( 'NONE', #113613, #54053, #124722 ) ;
#99108=CARTESIAN_POINT ( 'NONE',  ( 7.899999999999924860, 2.500000000000000000, 4.330127018922196314 ) ) ;
#99109=EDGE_LOOP ( 'NONE', ( #57038, #87468, #44360, #98093 ) ) ;
#99110=VERTEX_POINT ( 'NONE', #61749 ) ;
#99111=DIRECTION ( 'NONE',  ( -0.000000000000000000, 1.000000000000000000, -0.000000000000000000 ) ) ;
#99112=LINE ( 'NONE', #1534, #15875 ) ;
#99114=CARTESIAN_POINT ( 'NONE',  ( 1.649999999999951505, 12.50000000000000000, -2.857883832488653741 ) ) ;
#99115=FACE_OUTER_BOUND ( 'NONE', #90178, .T. ) ;
#99116=ORIENTED_EDGE ( 'NONE', *, *, #84747, .F. ) ;
#99117=AXIS2_PLACEMENT_3D ( 'NONE', #42673, #71447, #101572 ) ;
#99118=AXIS2_PLACEMENT_3D ( 'NONE', #112560, #22895, #62812 ) ;
#99119=CONICAL_SURFACE ( 'NONE', #80335, 0.1000000000000000472, 0.003490658503988666988 ) ;
#99120=CARTESIAN_POINT ( 'NONE',  ( -11.05000000000000249, 2.500000000000000000, -6.148780366869522673 ) ) ;
#99121=CIRCLE ( 'NONE', #46798, 0.1000000000000002554 ) ;
#99123=AXIS2_PLACEMENT_3D ( 'NONE', #21393, #103184, #91430 ) ;
#99126=DIRECTION ( 'NONE',  ( 0.000000000000000000, 0.000000000000000000, -1.000000000000000000 ) ) ;
#99127=CARTESIAN_POINT ( 'NONE',  ( -13.74999999999998757, 2.500000000000000000, -2.857883832488651521 ) ) ;
#99128=CARTESIAN_POINT ( 'NONE',  ( -4.550000000000026468, 2.500000000000000000, -6.495190528383302464 ) ) ;
#99129=FACE_OUTER_BOUND ( 'NONE', #60965, .T. ) ;
#99130=CARTESIAN_POINT ( 'NONE',  ( 0.4499999999999569344, 2.500000000000000000, 2.065063509461097624 ) ) ;
#99131=EDGE_LOOP ( 'NONE', ( #123137, #69276 ) ) ;
#99132=DIRECTION ( 'NONE',  ( 0.000000000000000000, -0.9999939076577903929, 0.003490651415223739937 ) ) ;
#99133=ADVANCED_FACE ( 'NONE', ( #91839 ), #81063, .T. ) ;
#99134=CARTESIAN_POINT ( 'NONE',  ( -9.400000000000007461, 12.50000000000000000, 4.676537180435972552 ) ) ;
#99135=PLANE ( 'NONE',  #129089 ) ;
#99136=AXIS2_PLACEMENT_3D ( 'NONE', #31798, #42264, #110972 ) ;
#99137=AXIS2_PLACEMENT_3D ( 'NONE', #5010, #84216, #35777 ) ;
#99138=ORIENTED_EDGE ( 'NONE', *, *, #35672, .F. ) ;
#99139=DIRECTION ( 'NONE',  ( 0.000000000000000000, -0.000000000000000000, 1.000000000000000000 ) ) ;
#99141=VECTOR ( 'NONE', #122343, 1000.000000000000000 ) ;
#99142=CIRCLE ( 'NONE', #44767, 0.09999999999999982514 ) ;
#99143=VERTEX_POINT ( 'NONE', #124526 ) ;
#99144=CIRCLE ( 'NONE', #42737, 0.06509327318403741736 ) ;
#99146=CARTESIAN_POINT ( 'NONE',  ( 13.34999999999990017, 2.500000000000000000, 1.472243186433545459 ) ) ;
#99147=VECTOR ( 'NONE', #91025, 1000.000000000000000 ) ;
#99148=ORIENTED_EDGE ( 'NONE', *, *, #127000, .F. ) ;
#99149=DIRECTION ( 'NONE',  ( 0.000000000000000000, 1.000000000000000000, 0.000000000000000000 ) ) ;
#99150=CARTESIAN_POINT ( 'NONE',  ( -4.076600168545496672E-14, 2.500000000000000000, -5.022947341949754119 ) ) ;
#99151=AXIS2_PLACEMENT_3D ( 'NONE', #112336, #120224, #30573 ) ;
#99153=CIRCLE ( 'NONE', #92902, 0.1000000000000002554 ) ;
#99154=CIRCLE ( 'NONE', #32276, 0.06509327318403745899 ) ;
#99155=DIRECTION ( 'NONE',  ( 0.000000000000000000, 1.000000000000000000, 0.000000000000000000 ) ) ;
#99156=DIRECTION ( 'NONE',  ( 0.000000000000000000, 0.000000000000000000, 1.000000000000000000 ) ) ;
#99157=ORIENTED_EDGE ( 'NONE', *, *, #40565, .F. ) ;
#99158=VECTOR ( 'NONE', #107295, 1000.000000000000000 ) ;
#99159=LINE ( 'NONE', #46839, #23498 ) ;
#99160=CARTESIAN_POINT ( 'NONE',  ( 12.49999999999990585, 12.50000000000000000, 3.637306695894644726 ) ) ;
#99161=EDGE_LOOP ( 'NONE', ( #8703, #23315 ) ) ;
#99162=ORIENTED_EDGE ( 'NONE', *, *, #16648, .T. ) ;
#99163=VERTEX_POINT ( 'NONE', #94397 ) ;
#99164=DIRECTION ( 'NONE',  ( 0.000000000000000000, 1.000000000000000000, 0.000000000000000000 ) ) ;
#99165=CARTESIAN_POINT ( 'NONE',  ( -12.49999999999995914, 12.50000000000000000, -4.330127018922198978 ) ) ;
#99166=DIRECTION ( 'NONE',  ( 0.000000000000000000, -0.000000000000000000, 1.000000000000000000 ) ) ;
#99167=FACE_BOUND ( 'NONE', #60663, .T. ) ;
#99168=ORIENTED_EDGE ( 'NONE', *, *, #57268, .F. ) ;
#99169=DIRECTION ( 'NONE',  ( 0.000000000000000000, 0.000000000000000000, 1.000000000000000000 ) ) ;
#99170=FACE_OUTER_BOUND ( 'NONE', #91489, .T. ) ;
#99171=CONICAL_SURFACE ( 'NONE', #97106, 0.1000000000000002554, 0.003490658503988666988 ) ;
#99172=VERTEX_POINT ( 'NONE', #105525 ) ;
#99173=LINE ( 'NONE', #109637, #105123 ) ;
#99175=DIRECTION ( 'NONE',  ( 0.000000000000000000, 0.000000000000000000, 1.000000000000000000 ) ) ;
#99176=CARTESIAN_POINT ( 'NONE',  ( 0.1999999999999636513, 12.50000000000000000, -0.4115034346978134749 ) ) ;
#99177=CARTESIAN_POINT ( 'NONE',  ( -12.89999999999999147, 2.500000000000000000, 4.430127018922196847 ) ) ;
#99178=DIRECTION ( 'NONE',  ( 0.000000000000000000, -0.9999939076577903929, 0.003490651415223739937 ) ) ;
#99179=DIRECTION ( 'NONE',  ( -0.000000000000000000, 1.000000000000000000, -0.000000000000000000 ) ) ;
#99180=FACE_OUTER_BOUND ( 'NONE', #14216, .T. ) ;
#99181=VECTOR ( 'NONE', #12236, 1000.000000000000000 ) ;
#99182=EDGE_CURVE ( 'NONE', #19500, #87143, #10046, .T. ) ;
#99183=CIRCLE ( 'NONE', #101335, 0.1000000000000002554 ) ;
#99184=ORIENTED_EDGE ( 'NONE', *, *, #794, .F. ) ;
#99185=ORIENTED_EDGE ( 'NONE', *, *, #47803, .F. ) ;
#99186=ORIENTED_EDGE ( 'NONE', *, *, #58314, .T. ) ;
#99187=ORIENTED_EDGE ( 'NONE', *, *, #551, .F. ) ;
#99188=ORIENTED_EDGE ( 'NONE', *, *, #5528, .F. ) ;
#99189=DIRECTION ( 'NONE',  ( 0.000000000000000000, 0.000000000000000000, -1.000000000000000000 ) ) ;
#99190=EDGE_CURVE ( 'NONE', #22979, #110935, #108237, .T. ) ;
#99191=CARTESIAN_POINT ( 'NONE',  ( 6.699999999999930012, 2.500000000000000000, 4.230127018922196669 ) ) ;
#99192=ORIENTED_EDGE ( 'NONE', *, *, #99412, .F. ) ;
#99193=FACE_BOUND ( 'NONE', #128645, .T. ) ;
#99194=EDGE_CURVE ( 'NONE', #15146, #43992, #63675, .T. ) ;
#99195=CARTESIAN_POINT ( 'NONE',  ( 7.499999999999927169, 2.500000000000000000, -5.022947341949754119 ) ) ;
#99196=CIRCLE ( 'NONE', #57330, 0.06509327318403745899 ) ;
#99197=EDGE_CURVE ( 'NONE', #92369, #15915, #83206, .T. ) ;
#99198=CARTESIAN_POINT ( 'NONE',  ( -4.550000000000022915, 2.500000000000000000, -2.165063509461101710 ) ) ;
#99199=CIRCLE ( 'NONE', #80422, 0.1000000000000002554 ) ;
#99200=CARTESIAN_POINT ( 'NONE',  ( -9.200000000000009948, 12.50000000000000000, -4.265033745738159965 ) ) ;
#99201=FACE_OUTER_BOUND ( 'NONE', #4948, .T. ) ;
#99202=CARTESIAN_POINT ( 'NONE',  ( -1.900000000000034550, 12.50000000000000000, 4.676537180435972552 ) ) ;
#99203=EDGE_CURVE ( 'NONE', #79720, #9937, #95726, .T. ) ;
#99204=DIRECTION ( 'NONE',  ( -0.000000000000000000, -1.000000000000000000, -0.000000000000000000 ) ) ;
#99205=VERTEX_POINT ( 'NONE', #55771 ) ;
#99206=ORIENTED_EDGE ( 'NONE', *, *, #121214, .F. ) ;
#99207=CONICAL_SURFACE ( 'NONE', #42799, 0.1000000000000002554, 0.003490658503988666988 ) ;
#99208=AXIS2_PLACEMENT_3D ( 'NONE', #90443, #72758, #51836 ) ;
#99209=EDGE_LOOP ( 'NONE', ( #49922, #104626 ) ) ;
#99210=ORIENTED_EDGE ( 'NONE', *, *, #5543, .T. ) ;
#99211=CARTESIAN_POINT ( 'NONE',  ( -9.350000000000008527, 12.50000000000000000, -6.841600689897072485 ) ) ;
#99212=DIRECTION ( 'NONE',  ( 0.000000000000000000, 0.000000000000000000, -1.000000000000000000 ) ) ;
#99213=AXIS2_PLACEMENT_3D ( 'NONE', #42045, #90474, #11280 ) ;
#99214=ORIENTED_EDGE ( 'NONE', *, *, #29805, .T. ) ;
#99215=DIRECTION ( 'NONE',  ( -0.000000000000000000, -1.000000000000000000, -0.000000000000000000 ) ) ;
#99216=AXIS2_PLACEMENT_3D ( 'NONE', #127972, #78896, #86755 ) ;
#99217=DIRECTION ( 'NONE',  ( 0.000000000000000000, 0.000000000000000000, -1.000000000000000000 ) ) ;
#99218=DIRECTION ( 'NONE',  ( 0.000000000000000000, 0.000000000000000000, 1.000000000000000000 ) ) ;
#99220=CARTESIAN_POINT ( 'NONE',  ( -3.950000000000028155, 2.500000000000000000, -6.841600689897077814 ) ) ;
#99221=DIRECTION ( 'NONE',  ( 0.000000000000000000, -0.000000000000000000, 1.000000000000000000 ) ) ;
#99222=CARTESIAN_POINT ( 'NONE',  ( 5.649999999999932854, 12.50000000000000000, 2.511473670974873507 ) ) ;
#99223=ORIENTED_EDGE ( 'NONE', *, *, #89206, .T. ) ;
#99224=CARTESIAN_POINT ( 'NONE',  ( -5.800000000000022027, 2.500000000000000000, -4.330127018922201643 ) ) ;
#99225=ORIENTED_EDGE ( 'NONE', *, *, #93730, .F. ) ;
#99226=EDGE_CURVE ( 'NONE', #38808, #76595, #28830, .T. ) ;
#99227=AXIS2_PLACEMENT_3D ( 'NONE', #86356, #7802, #127588 ) ;
#99228=ORIENTED_EDGE ( 'NONE', *, *, #77240, .T. ) ;
#99229=DIRECTION ( 'NONE',  ( -0.000000000000000000, 1.000000000000000000, -0.000000000000000000 ) ) ;
#99230=CONICAL_SURFACE ( 'NONE', #65756, 0.1000000000000002554, 0.003490658503988666988 ) ;
#99231=CONICAL_SURFACE ( 'NONE', #36545, 0.1000000000000002554, 0.003490658503988666988 ) ;
#99232=DIRECTION ( 'NONE',  ( 0.000000000000000000, 1.000000000000000000, 0.000000000000000000 ) ) ;
#99233=CONICAL_SURFACE ( 'NONE', #72044, 0.09999999999999982514, 0.003490658503988666988 ) ;
#99234=DIRECTION ( 'NONE',  ( 0.000000000000000000, 0.000000000000000000, 1.000000000000000000 ) ) ;
#99235=ORIENTED_EDGE ( 'NONE', *, *, #82832, .F. ) ;
#99236=ORIENTED_EDGE ( 'NONE', *, *, #33728, .T. ) ;
#99237=EDGE_CURVE ( 'NONE', #113231, #2251, #83117, .T. ) ;
#99238=DIRECTION ( 'NONE',  ( 0.000000000000000000, 0.000000000000000000, -1.000000000000000000 ) ) ;
#99239=CONICAL_SURFACE ( 'NONE', #84559, 0.09999999999999982514, 0.003490658503988666988 ) ;
#99240=AXIS2_PLACEMENT_3D ( 'NONE', #15630, #126899, #73926 ) ;
#99241=CIRCLE ( 'NONE', #67922, 0.09999999999999982514 ) ;
#99242=LINE ( 'NONE', #69766, #1433 ) ;
#99243=CARTESIAN_POINT ( 'NONE',  ( 12.93920187831609603, -1.500000000000000000, -9.999999999999998224 ) ) ;
#99244=VERTEX_POINT ( 'NONE', #106168 ) ;
#99245=EDGE_CURVE ( 'NONE', #33099, #96862, #55991, .T. ) ;
#99246=AXIS2_PLACEMENT_3D ( 'NONE', #110539, #41825, #40540 ) ;
#99247=DIRECTION ( 'NONE',  ( 0.000000000000000000, -0.9999939076577903929, 0.003490651415223739937 ) ) ;
#99248=EDGE_CURVE ( 'NONE', #38209, #58662, #16269, .T. ) ;
#99249=ADVANCED_FACE ( 'NONE', ( #15837 ), #104127, .T. ) ;
#99250=ORIENTED_EDGE ( 'NONE', *, *, #114857, .T. ) ;
#99251=DIRECTION ( 'NONE',  ( 0.000000000000000000, 0.000000000000000000, -1.000000000000000000 ) ) ;
#99252=AXIS2_PLACEMENT_3D ( 'NONE', #41008, #80910, #21330 ) ;
#99253=CIRCLE ( 'NONE', #17656, 0.06509327318403745899 ) ;
#99254=EDGE_LOOP ( 'NONE', ( #76995, #49333, #117212, #33996 ) ) ;
#99256=ADVANCED_FACE ( 'NONE', ( #95707 ), #129284, .T. ) ;
#99257=CARTESIAN_POINT ( 'NONE',  ( -11.84999999999999609, 12.50000000000000000, 6.148780366869520897 ) ) ;
#99258=DIRECTION ( 'NONE',  ( -0.000000000000000000, -1.000000000000000000, -0.000000000000000000 ) ) ;
#99259=CIRCLE ( 'NONE', #101306, 0.09999999999999982514 ) ;
#99260=DIRECTION ( 'NONE',  ( 0.000000000000000000, 0.000000000000000000, -1.000000000000000000 ) ) ;
#99261=ORIENTED_EDGE ( 'NONE', *, *, #6555, .T. ) ;
#99262=EDGE_CURVE ( 'NONE', #48101, #61538, #5897, .T. ) ;
#99263=CARTESIAN_POINT ( 'NONE',  ( -13.09999999999999254, 2.500000000000000000, -4.083716857408424161 ) ) ;
#99264=EDGE_CURVE ( 'NONE', #113868, #8077, #56409, .T. ) ;
#99265=ORIENTED_EDGE ( 'NONE', *, *, #65847, .T. ) ;
#99266=ORIENTED_EDGE ( 'NONE', *, *, #23169, .T. ) ;
#99267=CARTESIAN_POINT ( 'NONE',  ( 1.249999999999952482, 2.500000000000000000, -5.702370205355749455 ) ) ;
#99268=FACE_OUTER_BOUND ( 'NONE', #52819, .T. ) ;
#99269=LINE ( 'NONE', #10846, #67856 ) ;
#99270=DIRECTION ( 'NONE',  ( 0.000000000000000000, 0.000000000000000000, 1.000000000000000000 ) ) ;
#99271=CONICAL_SURFACE ( 'NONE', #51153, 0.1000000000000002554, 0.003490658503988666988 ) ;
#99272=DIRECTION ( 'NONE',  ( -0.000000000000000000, -1.000000000000000000, -0.000000000000000000 ) ) ;
#99273=CARTESIAN_POINT ( 'NONE',  ( 7.699999999999923794, 12.50000000000000000, 4.676537180435972552 ) ) ;
#99274=CARTESIAN_POINT ( 'NONE',  ( 5.849999999999933920, 2.500000000000000000, -2.265063509461101798 ) ) ;
#99275=LINE ( 'NONE', #9596, #122333 ) ;
#99276=LINE ( 'NONE', #60011, #4554 ) ;
#99277=CIRCLE ( 'NONE', #9390, 0.06509327318403745899 ) ;
#99278=VERTEX_POINT ( 'NONE', #104856 ) ;
#99279=DIRECTION ( 'NONE',  ( 0.000000000000000000, 0.000000000000000000, 1.000000000000000000 ) ) ;
#99280=DIRECTION ( 'NONE',  ( -4.274815082592931898E-19, -0.9999939076577903929, -0.003490651415223739937 ) ) ;
#99281=DIRECTION ( 'NONE',  ( 0.000000000000000000, 0.000000000000000000, 1.000000000000000000 ) ) ;
#99282=DIRECTION ( 'NONE',  ( 0.000000000000000000, 0.000000000000000000, -1.000000000000000000 ) ) ;
#99283=DIRECTION ( 'NONE',  ( -0.000000000000000000, 1.000000000000000000, -0.000000000000000000 ) ) ;
#99285=CARTESIAN_POINT ( 'NONE',  ( -5.000000000000022204, 2.500000000000000000, -0.6928203230275541413 ) ) ;
#99286=CIRCLE ( 'NONE', #51173, 0.06509327318403745899 ) ;
#99287=EDGE_CURVE ( 'NONE', #77185, #89102, #72833, .T. ) ;
#99288=CONICAL_SURFACE ( 'NONE', #109751, 0.09999999999999982514, 0.003490658503988666988 ) ;
#99289=CARTESIAN_POINT ( 'NONE',  ( -9.350000000000008527, 12.50000000000000000, -6.148780366869520897 ) ) ;
#99290=FACE_OUTER_BOUND ( 'NONE', #6024, .T. ) ;
#99291=VERTEX_POINT ( 'NONE', #36140 ) ;
#99292=EDGE_LOOP ( 'NONE', ( #53313, #108167 ) ) ;
#99293=CARTESIAN_POINT ( 'NONE',  ( 9.149999999999915090, 12.50000000000000000, -2.165063509461101710 ) ) ;
#99294=ADVANCED_FACE ( 'NONE', ( #6012 ), #114573, .T. ) ;
#99295=CIRCLE ( 'NONE', #49136, 0.09999999999999982514 ) ;
#99296=AXIS2_PLACEMENT_3D ( 'NONE', #46074, #125274, #124630 ) ;
#99297=EDGE_LOOP ( 'NONE', ( #52572, #84663, #37563, #105134 ) ) ;
#99298=EDGE_LOOP ( 'NONE', ( #108272, #80548 ) ) ;
#99299=ORIENTED_EDGE ( 'NONE', *, *, #117361, .F. ) ;
#99300=DIRECTION ( 'NONE',  ( 0.000000000000000000, 1.000000000000000000, 0.000000000000000000 ) ) ;
#99301=CARTESIAN_POINT ( 'NONE',  ( 19.40342015654704610, 2.551666867760210788, -4.359384978532800936 ) ) ;
#99302=LINE ( 'NONE', #20094, #102653 ) ;
#99303=DIRECTION ( 'NONE',  ( 0.000000000000000000, 0.000000000000000000, -1.000000000000000000 ) ) ;
#99304=ORIENTED_EDGE ( 'NONE', *, *, #26082, .T. ) ;
#99305=CARTESIAN_POINT ( 'NONE',  ( 4.399999999999937295, 2.500000000000000000, 4.676537180435972552 ) ) ;
#99306=EDGE_LOOP ( 'NONE', ( #93600, #117825, #25354, #88036 ) ) ;
#99307=CARTESIAN_POINT ( 'NONE',  ( 3.549999999999941203, 12.50000000000000000, 6.148780366869520897 ) ) ;
#99308=DIRECTION ( 'NONE',  ( 0.000000000000000000, 0.000000000000000000, 1.000000000000000000 ) ) ;
#99309=LINE ( 'NONE', #37805, #63121 ) ;
#99310=CARTESIAN_POINT ( 'NONE',  ( -5.850000000000018296, 2.500000000000000000, 2.857883832488649301 ) ) ;
#99311=AXIS2_PLACEMENT_3D ( 'NONE', #60299, #51112, #121121 ) ;
#99312=EDGE_LOOP ( 'NONE', ( #103606, #59642 ) ) ;
#99313=AXIS2_PLACEMENT_3D ( 'NONE', #120764, #80204, #21264 ) ;
#99314=ORIENTED_EDGE ( 'NONE', *, *, #16335, .T. ) ;
#99315=ORIENTED_EDGE ( 'NONE', *, *, #107139, .F. ) ;
#99316=AXIS2_PLACEMENT_3D ( 'NONE', #17960, #19235, #48083 ) ;
#99317=VERTEX_POINT ( 'NONE', #58370 ) ;
#99318=ORIENTED_EDGE ( 'NONE', *, *, #120762, .F. ) ;
#99319=CARTESIAN_POINT ( 'NONE',  ( -0.2000000000000408673, 2.500000000000000000, -3.883716857408426648 ) ) ;
#99320=CARTESIAN_POINT ( 'NONE',  ( -5.850000000000022737, 2.500000000000000000, -6.495190528383302464 ) ) ;
#99321=VECTOR ( 'NONE', #85201, 1000.000000000000000 ) ;
#99322=DIRECTION ( 'NONE',  ( -0.000000000000000000, 1.000000000000000000, -0.000000000000000000 ) ) ;
#99323=FACE_BOUND ( 'NONE', #126902, .T. ) ;
#99324=CARTESIAN_POINT ( 'NONE',  ( -10.85000000000000142, 2.500000000000000000, 6.395190528383296602 ) ) ;
#99325=DIRECTION ( 'NONE',  ( 0.000000000000000000, -0.9999939076577903929, 0.003490651415223739937 ) ) ;
#99326=PLANE ( 'NONE',  #30176 ) ;
#99327=DIRECTION ( 'NONE',  ( -0.000000000000000000, -1.000000000000000000, -0.000000000000000000 ) ) ;
#99328=AXIS2_PLACEMENT_3D ( 'NONE', #97308, #114992, #104547 ) ;
#99329=CIRCLE ( 'NONE', #42824, 0.09999999999999982514 ) ;
#99330=VECTOR ( 'NONE', #67019, 1000.000000000000000 ) ;
#99331=DIRECTION ( 'NONE',  ( 0.000000000000000000, 0.000000000000000000, 1.000000000000000000 ) ) ;
#99332=AXIS2_PLACEMENT_3D ( 'NONE', #80293, #79016, #31202 ) ;
#99333=DIRECTION ( 'NONE',  ( 0.000000000000000000, 1.000000000000000000, 0.000000000000000000 ) ) ;
#99334=DIRECTION ( 'NONE',  ( -0.000000000000000000, -1.000000000000000000, -0.000000000000000000 ) ) ;
#99335=CIRCLE ( 'NONE', #93077, 0.06509327318403745899 ) ;
#99336=VECTOR ( 'NONE', #106580, 1000.000000000000000 ) ;
#99337=EDGE_CURVE ( 'NONE', #11600, #97446, #87382, .T. ) ;
#99338=CARTESIAN_POINT ( 'NONE',  ( -10.40000000000000213, 2.500000000000000000, -4.230127018922197557 ) ) ;
#99339=ORIENTED_EDGE ( 'NONE', *, *, #128407, .F. ) ;
#99340=ORIENTED_EDGE ( 'NONE', *, *, #70021, .F. ) ;
#99341=ORIENTED_EDGE ( 'NONE', *, *, #98017, .F. ) ;
#99343=CIRCLE ( 'NONE', #42932, 0.06509327318403745899 ) ;
#99344=CARTESIAN_POINT ( 'NONE',  ( -4.400000000000025224, 12.50000000000000000, 3.983716857408420076 ) ) ;
#99345=EDGE_CURVE ( 'NONE', #59160, #28644, #47701, .T. ) ;
#99346=DIRECTION ( 'NONE',  ( 0.000000000000000000, 0.000000000000000000, 1.000000000000000000 ) ) ;
#99347=FACE_BOUND ( 'NONE', #73757, .T. ) ;
#99348=EDGE_CURVE ( 'NONE', #93851, #37658, #116617, .T. ) ;
#99349=FACE_OUTER_BOUND ( 'NONE', #101329, .T. ) ;
#99350=EDGE_CURVE ( 'NONE', #121936, #64779, #62378, .T. ) ;
#99351=EDGE_CURVE ( 'NONE', #126997, #79185, #3781, .T. ) ;
#99352=ORIENTED_EDGE ( 'NONE', *, *, #72588, .F. ) ;
#99353=CARTESIAN_POINT ( 'NONE',  ( -0.8500000000000390576, 2.500000000000000000, -6.395190528383301931 ) ) ;
#99355=DIRECTION ( 'NONE',  ( 0.000000000000000000, 0.000000000000000000, -1.000000000000000000 ) ) ;
#99356=ADVANCED_FACE ( 'NONE', ( #120979 ), #127730, .T. ) ;
#99357=CARTESIAN_POINT ( 'NONE',  ( 11.69999999999990870, 2.500000000000000000, 4.330127018922196314 ) ) ;
#99358=VECTOR ( 'NONE', #90473, 1000.000000000000000 ) ;
#99359=EDGE_LOOP ( 'NONE', ( #63371, #92742, #57307, #103038 ) ) ;
#99360=CARTESIAN_POINT ( 'NONE',  ( -10.00000000000000355, 2.500000000000000000, -0.6928203230275541413 ) ) ;
#99361=EDGE_LOOP ( 'NONE', ( #119292, #56929, #28110, #125169 ) ) ;
#99362=ORIENTED_EDGE ( 'NONE', *, *, #11478, .F. ) ;
#99363=CARTESIAN_POINT ( 'NONE',  ( 10.44999999999991402, 12.50000000000000000, -2.099970236277064473 ) ) ;
#99364=CARTESIAN_POINT ( 'NONE',  ( -6.050000000000017586, 2.500000000000000000, 6.248780366869520542 ) ) ;
#99365=AXIS2_PLACEMENT_3D ( 'NONE', #15790, #95016, #43988 ) ;
#99366=ORIENTED_EDGE ( 'NONE', *, *, #2360, .F. ) ;
#99367=CIRCLE ( 'NONE', #3224, 0.06509327318403745899 ) ;
#99368=AXIS2_PLACEMENT_3D ( 'NONE', #57316, #127353, #87400 ) ;
#99369=LINE ( 'NONE', #69234, #78212 ) ;
#99370=CARTESIAN_POINT ( 'NONE',  ( 8.349999999999923261, 2.500000000000000000, -7.288010851410854585 ) ) ;
#99371=ORIENTED_EDGE ( 'NONE', *, *, #19046, .F. ) ;
#99372=DIRECTION ( 'NONE',  ( 0.000000000000000000, -0.000000000000000000, 1.000000000000000000 ) ) ;
#99373=ORIENTED_EDGE ( 'NONE', *, *, #100518, .T. ) ;
#99374=CARTESIAN_POINT ( 'NONE',  ( 11.84999999999990727, 12.50000000000000000, 6.841600689897072485 ) ) ;
#99375=EDGE_LOOP ( 'NONE', ( #14035, #59386 ) ) ;
#99376=CARTESIAN_POINT ( 'NONE',  ( 7.949999999999922018, 12.50000000000000000, -2.165063509461101710 ) ) ;
#99377=FACE_BOUND ( 'NONE', #63596, .T. ) ;
#99378=CIRCLE ( 'NONE', #51278, 0.1000000000000000472 ) ;
#99379=ORIENTED_EDGE ( 'NONE', *, *, #82059, .F. ) ;
#99380=AXIS2_PLACEMENT_3D ( 'NONE', #54114, #34495, #114320 ) ;
#99382=ORIENTED_EDGE ( 'NONE', *, *, #86413, .F. ) ;
#99384=CARTESIAN_POINT ( 'NONE',  ( -8.100000000000013856, 12.50000000000000000, 0.2813168883297362810 ) ) ;
#99385=DIRECTION ( 'NONE',  ( 0.000000000000000000, -0.000000000000000000, 1.000000000000000000 ) ) ;
#99386=CARTESIAN_POINT ( 'NONE',  ( 10.39999999999991154, 12.50000000000000000, 3.702399969078682407 ) ) ;
#99387=CARTESIAN_POINT ( 'NONE',  ( -12.69999999999999396, 12.50000000000000000, 0.2813168883297402778 ) ) ;
#99388=VERTEX_POINT ( 'NONE', #87155 ) ;
#99389=VERTEX_POINT ( 'NONE', #76704 ) ;
#99391=DIRECTION ( 'NONE',  ( 0.000000000000000000, 0.000000000000000000, 1.000000000000000000 ) ) ;
#99392=VECTOR ( 'NONE', #9366, 1000.000000000000000 ) ;
#99393=DIRECTION ( 'NONE',  ( 0.000000000000000000, 0.000000000000000000, -1.000000000000000000 ) ) ;
#99394=DIRECTION ( 'NONE',  ( -0.000000000000000000, 1.000000000000000000, -0.000000000000000000 ) ) ;
#99395=EDGE_CURVE ( 'NONE', #15286, #31758, #1709, .T. ) ;
#99396=ORIENTED_EDGE ( 'NONE', *, *, #5784, .T. ) ;
#99397=VERTEX_POINT ( 'NONE', #106791 ) ;
#99398=VERTEX_POINT ( 'NONE', #71225 ) ;
#99399=EDGE_CURVE ( 'NONE', #62733, #30373, #60237, .T. ) ;
#99400=DIRECTION ( 'NONE',  ( 0.000000000000000000, -0.000000000000000000, 1.000000000000000000 ) ) ;
#99401=EDGE_CURVE ( 'NONE', #64551, #23628, #20517, .T. ) ;
#99404=DIRECTION ( 'NONE',  ( 0.000000000000000000, 0.000000000000000000, 1.000000000000000000 ) ) ;
#99405=CARTESIAN_POINT ( 'NONE',  ( -6.900000000000019007, 2.500000000000000000, -4.776537180435978414 ) ) ;
#99406=CIRCLE ( 'NONE', #53431, 0.09999999999999982514 ) ;
#99407=DIRECTION ( 'NONE',  ( 0.000000000000000000, 1.000000000000000000, 0.000000000000000000 ) ) ;
#99408=B_SPLINE_CURVE_WITH_KNOTS ( 'NONE', 3,
 ( #59298, #88735, #96599, #118196, #87434, #98531, #18697, #9536, #129333, #49477, #89386, #76983, #29820, #108370, #116885, #128016, #39663, #109672, #27228, #79567 ),
 .UNSPECIFIED., .F., .F.,
 ( 4, 2, 2, 2, 2, 2, 2, 2, 2, 4 ),
 ( 0.000000000000000000, 0.003515823931524271733, 0.005273735897286407383, 0.007031647863048543466, 0.008789559828810680417, 0.01054747179457281477, 0.01142642777745388021, 0.01230538376033494564, 0.01318433974321600935, 0.01406329572609707479 ),
 .UNSPECIFIED. ) ;
#99409=DIRECTION ( 'NONE',  ( -4.274815082592931898E-19, -0.9999939076577903929, -0.003490651415223739937 ) ) ;
#99410=LINE ( 'NONE', #20842, #61298 ) ;
#99411=EDGE_CURVE ( 'NONE', #113868, #26724, #125048, .T. ) ;
#99412=EDGE_CURVE ( 'NONE', #10651, #76320, #43507, .T. ) ;
#99413=CONICAL_SURFACE ( 'NONE', #42992, 0.1000000000000002554, 0.003490658503988666988 ) ;
#99414=CARTESIAN_POINT ( 'NONE',  ( 2.899999999999946620, 2.500000000000000000, -4.922947341949753586 ) ) ;
#99415=EDGE_CURVE ( 'NONE', #49108, #127376, #95808, .T. ) ;
#99416=ORIENTED_EDGE ( 'NONE', *, *, #112188, .T. ) ;
#99417=ADVANCED_FACE ( 'NONE', ( #120341 ), #14225, .T. ) ;
#99418=EDGE_LOOP ( 'NONE', ( #4686, #93673, #116864, #20188 ) ) ;
#99419=DIRECTION ( 'NONE',  ( 0.000000000000000000, 0.000000000000000000, -1.000000000000000000 ) ) ;
#99420=ADVANCED_FACE ( 'NONE', ( #1201 ), #106274, .T. ) ;
#99421=VECTOR ( 'NONE', #98373, 1000.000000000000000 ) ;
#99422=AXIS2_PLACEMENT_3D ( 'NONE', #66257, #68840, #127763 ) ;
#99423=DIRECTION ( 'NONE',  ( 0.000000000000000000, 0.000000000000000000, 1.000000000000000000 ) ) ;
#99424=ORIENTED_EDGE ( 'NONE', *, *, #24198, .T. ) ;
#99425=ORIENTED_EDGE ( 'NONE', *, *, #36207, .T. ) ;
#99427=DIRECTION ( 'NONE',  ( 0.000000000000000000, 0.000000000000000000, 1.000000000000000000 ) ) ;
#99428=CARTESIAN_POINT ( 'NONE',  ( 2.500000000000002220, 2.500000000000000000, -9.261799387799149130 ) ) ;
#99430=AXIS2_PLACEMENT_3D ( 'NONE', #107453, #6632, #58373 ) ;
#99431=DIRECTION ( 'NONE',  ( -4.274815082592931898E-19, -0.9999939076577903929, -0.003490651415223739937 ) ) ;
#99432=DIRECTION ( 'NONE',  ( -0.000000000000000000, -1.000000000000000000, -0.000000000000000000 ) ) ;
#99433=DIRECTION ( 'NONE',  ( 0.000000000000000000, -0.000000000000000000, 1.000000000000000000 ) ) ;
#99434=CARTESIAN_POINT ( 'NONE',  ( -12.49999999999999467, 12.50000000000000000, -3.637306695894647390 ) ) ;
#99435=CONICAL_SURFACE ( 'NONE', #84746, 0.1000000000000000056, 0.003490658503988666988 ) ;
#99436=DIRECTION ( 'NONE',  ( 0.000000000000000000, 0.000000000000000000, 1.000000000000000000 ) ) ;
#99437=AXIS2_PLACEMENT_3D ( 'NONE', #40854, #21179, #29093 ) ;
#99438=AXIS2_PLACEMENT_3D ( 'NONE', #77456, #26432, #27701 ) ;
#99439=ORIENTED_EDGE ( 'NONE', *, *, #86693, .T. ) ;
#99440=CONICAL_SURFACE ( 'NONE', #59737, 0.1000000000000000472, 0.003490658503988666988 ) ;
#99441=ORIENTED_EDGE ( 'NONE', *, *, #122929, .T. ) ;
#99442=AXIS2_PLACEMENT_3D ( 'NONE', #65450, #123099, #64166 ) ;
#99443=ORIENTED_EDGE ( 'NONE', *, *, #39975, .T. ) ;
#99444=VERTEX_POINT ( 'NONE', #50965 ) ;
#99445=CARTESIAN_POINT ( 'NONE',  ( 14.34999999999989306, 2.500000000000000000, -1.818653347947326138 ) ) ;
#99446=LINE ( 'NONE', #47760, #1933 ) ;
#99447=VERTEX_POINT ( 'NONE', #41150 ) ;
#99448=LINE ( 'NONE', #573, #44485 ) ;
#99449=DIRECTION ( 'NONE',  ( -0.000000000000000000, -1.000000000000000000, -0.000000000000000000 ) ) ;
#99450=DIRECTION ( 'NONE',  ( -0.000000000000000000, 1.000000000000000000, -0.000000000000000000 ) ) ;
#99451=CARTESIAN_POINT ( 'NONE',  ( 6.899999999999928413, 12.50000000000000000, -4.741630453620015118 ) ) ;
#99452=ORIENTED_EDGE ( 'NONE', *, *, #22996, .F. ) ;
#99453=DIRECTION ( 'NONE',  ( -4.274815082592931898E-19, -0.9999939076577903929, -0.003490651415223739937 ) ) ;
#99454=VECTOR ( 'NONE', #106108, 1000.000000000000000 ) ;
#99455=CARTESIAN_POINT ( 'NONE',  ( 6.249999999999930722, 2.500000000000000000, 1.572243186433545548 ) ) ;
#99456=ORIENTED_EDGE ( 'NONE', *, *, #2414, .F. ) ;
#99457=EDGE_CURVE ( 'NONE', #88690, #37178, #37241, .T. ) ;
#99458=ORIENTED_EDGE ( 'NONE', *, *, #14249, .T. ) ;
#99459=EDGE_LOOP ( 'NONE', ( #36827, #38171 ) ) ;
#99460=ORIENTED_EDGE ( 'NONE', *, *, #37170, .F. ) ;
#99461=FACE_OUTER_BOUND ( 'NONE', #34613, .T. ) ;
#99462=AXIS2_PLACEMENT_3D ( 'NONE', #70060, #11118, #9848 ) ;
#99463=AXIS2_PLACEMENT_3D ( 'NONE', #45413, #85321, #40098 ) ;
#99464=DIRECTION ( 'NONE',  ( 0.000000000000000000, 0.000000000000000000, -1.000000000000000000 ) ) ;
#99465=DIRECTION ( 'NONE',  ( 0.000000000000000000, 1.000000000000000000, 0.000000000000000000 ) ) ;
#99466=CIRCLE ( 'NONE', #80678, 0.1000000000000002554 ) ;
#99467=ORIENTED_EDGE ( 'NONE', *, *, #69369, .T. ) ;
#99468=DIRECTION ( 'NONE',  ( 0.000000000000000000, -0.9999939076577903929, 0.003490651415223739937 ) ) ;
#99469=CARTESIAN_POINT ( 'NONE',  ( -6.250000000000017764, 2.500000000000000000, 2.957883832488649389 ) ) ;
#99470=ADVANCED_FACE ( 'NONE', ( #18426 ), #85344, .T. ) ;
#99471=DIRECTION ( 'NONE',  ( 0.000000000000000000, 0.000000000000000000, 1.000000000000000000 ) ) ;
#99472=FACE_OUTER_BOUND ( 'NONE', #60371, .T. ) ;
#99473=CIRCLE ( 'NONE', #38857, 0.06509327318403745899 ) ;
#99474=ORIENTED_EDGE ( 'NONE', *, *, #101444, .T. ) ;
#99476=CIRCLE ( 'NONE', #91151, 0.06509327318403745899 ) ;
#99477=CONICAL_SURFACE ( 'NONE', #89002, 0.09999999999999999167, 0.003490658503988666988 ) ;
#99478=ORIENTED_EDGE ( 'NONE', *, *, #93037, .T. ) ;
#99479=ORIENTED_EDGE ( 'NONE', *, *, #91612, .F. ) ;
#99480=DIRECTION ( 'NONE',  ( -0.000000000000000000, 1.000000000000000000, -0.000000000000000000 ) ) ;
#99481=CARTESIAN_POINT ( 'NONE',  ( 5.599999999999933031, 2.500000000000000000, 0.4464101615137735513 ) ) ;
#99482=FACE_BOUND ( 'NONE', #86419, .T. ) ;
#99483=DIRECTION ( 'NONE',  ( 0.000000000000000000, -0.000000000000000000, 1.000000000000000000 ) ) ;
#99484=DIRECTION ( 'NONE',  ( 0.000000000000000000, 0.000000000000000000, 1.000000000000000000 ) ) ;
#99485=DIRECTION ( 'NONE',  ( -4.274815082592931898E-19, -0.9999939076577903929, -0.003490651415223739937 ) ) ;
#99486=AXIS2_PLACEMENT_3D ( 'NONE', #19812, #67600, #59094 ) ;
#99488=VERTEX_POINT ( 'NONE', #111813 ) ;
#99489=CARTESIAN_POINT ( 'NONE',  ( 5.649999999999932854, 2.500000000000000000, 2.611473670974873151 ) ) ;
#99490=DIRECTION ( 'NONE',  ( 0.000000000000000000, 1.000000000000000000, 0.000000000000000000 ) ) ;
#99491=DIRECTION ( 'NONE',  ( -4.274815082592931898E-19, -0.9999939076577903929, -0.003490651415223739937 ) ) ;
#99492=FACE_OUTER_BOUND ( 'NONE', #572, .T. ) ;
#99493=ORIENTED_EDGE ( 'NONE', *, *, #114393, .T. ) ;
#99494=DIRECTION ( 'NONE',  ( -0.000000000000000000, 1.000000000000000000, -0.000000000000000000 ) ) ;
#99495=EDGE_CURVE ( 'NONE', #129161, #44450, #56089, .T. ) ;
#99496=FACE_OUTER_BOUND ( 'NONE', #33369, .T. ) ;
#99497=VERTEX_POINT ( 'NONE', #24715 ) ;
#99498=VERTEX_POINT ( 'NONE', #121609 ) ;
#99499=FACE_OUTER_BOUND ( 'NONE', #116767, .T. ) ;
#99500=CARTESIAN_POINT ( 'NONE',  ( 2.499999999999983569, 12.50000000000000000, -0.06509327318403970719 ) ) ;
#99501=FACE_BOUND ( 'NONE', #125032, .T. ) ;
#99502=EDGE_CURVE ( 'NONE', #27192, #127834, #41459, .T. ) ;
#99503=DIRECTION ( 'NONE',  ( 0.000000000000000000, 1.000000000000000000, 0.000000000000000000 ) ) ;
#99504=AXIS2_PLACEMENT_3D ( 'NONE', #43363, #65556, #34838 ) ;
#99505=DIRECTION ( 'NONE',  ( 0.000000000000000000, 1.000000000000000000, 0.000000000000000000 ) ) ;
#99506=AXIS2_PLACEMENT_3D ( 'NONE', #22338, #92337, #79947 ) ;
#99507=ADVANCED_FACE ( 'NONE', ( #104557 ), #82361, .T. ) ;
#99508=EDGE_CURVE ( 'NONE', #41415, #95053, #127127, .T. ) ;
#99510=EDGE_LOOP ( 'NONE', ( #57106, #24944 ) ) ;
#99511=DIRECTION ( 'NONE',  ( 0.000000000000000000, 0.000000000000000000, 1.000000000000000000 ) ) ;
#99512=ADVANCED_FACE ( 'NONE', ( #22158 ), #58598, .T. ) ;
#99513=EDGE_CURVE ( 'NONE', #116043, #85535, #10131, .T. ) ;
#99515=EDGE_CURVE ( 'NONE', #54777, #66462, #94094, .T. ) ;
#99516=EDGE_LOOP ( 'NONE', ( #17248, #70480, #82446, #91095 ) ) ;
#99517=LINE ( 'NONE', #97560, #854 ) ;
#99518=CARTESIAN_POINT ( 'NONE',  ( -11.44999999999999751, 2.500000000000000000, -2.611473670974873595 ) ) ;
#99519=VECTOR ( 'NONE', #45088, 1000.000000000000000 ) ;
#99520=CARTESIAN_POINT ( 'NONE',  ( 6.049999999999934097, 2.500000000000000000, -6.248780366869526759 ) ) ;
#99522=CONICAL_SURFACE ( 'NONE', #74474, 0.1000000000000002554, 0.003490658503988666988 ) ;
#99523=ADVANCED_FACE ( 'NONE', ( #86179 ), #26853, .T. ) ;
#99524=ORIENTED_EDGE ( 'NONE', *, *, #41158, .T. ) ;
#99525=CONICAL_SURFACE ( 'NONE', #97456, 0.09999999999999982514, 0.003490658503988666988 ) ;
#99526=DIRECTION ( 'NONE',  ( 0.000000000000000000, 0.000000000000000000, 1.000000000000000000 ) ) ;
#99527=CARTESIAN_POINT ( 'NONE',  ( -3.550000000000027356, 2.500000000000000000, 1.818653347947321475 ) ) ;
#99528=CARTESIAN_POINT ( 'NONE',  ( -0.6000000000000383915, 12.50000000000000000, -3.983716857408426293 ) ) ;
#99529=AXIS2_PLACEMENT_3D ( 'NONE', #17639, #57591, #48401 ) ;
#99530=DIRECTION ( 'NONE',  ( 0.000000000000000000, 0.000000000000000000, 1.000000000000000000 ) ) ;
#99531=ORIENTED_EDGE ( 'NONE', *, *, #120108, .F. ) ;
#99532=ORIENTED_EDGE ( 'NONE', *, *, #2264, .F. ) ;
#99534=ORIENTED_EDGE ( 'NONE', *, *, #5049, .T. ) ;
#99535=LINE ( 'NONE', #109990, #17940 ) ;
#99536=FACE_OUTER_BOUND ( 'NONE', #21648, .T. ) ;
#99537=DIRECTION ( 'NONE',  ( 0.000000000000000000, 1.000000000000000000, 0.000000000000000000 ) ) ;
#99538=ORIENTED_EDGE ( 'NONE', *, *, #104849, .F. ) ;
#99539=LINE ( 'NONE', #78618, #62168 ) ;
#99540=CARTESIAN_POINT ( 'NONE',  ( 5.199999999999931788, 2.500000000000000000, 4.776537180435972196 ) ) ;
#99541=DIRECTION ( 'NONE',  ( 0.000000000000000000, 0.000000000000000000, 1.000000000000000000 ) ) ;
#99542=CARTESIAN_POINT ( 'NONE',  ( -0.6500000000000394351, 2.500000000000000000, 2.511473670974873507 ) ) ;
#99543=CARTESIAN_POINT ( 'NONE',  ( 0.1999999999999636513, 12.50000000000000000, -0.2813168883297386680 ) ) ;
#99544=CONICAL_SURFACE ( 'NONE', #57683, 0.1000000000000002554, 0.003490658503988666988 ) ;
#99545=DIRECTION ( 'NONE',  ( 0.000000000000000000, 1.000000000000000000, 0.000000000000000000 ) ) ;
#99546=ORIENTED_EDGE ( 'NONE', *, *, #45971, .T. ) ;
#99547=ORIENTED_EDGE ( 'NONE', *, *, #56326, .F. ) ;
#99548=DIRECTION ( 'NONE',  ( 0.000000000000000000, 0.000000000000000000, -1.000000000000000000 ) ) ;
#99549=VERTEX_POINT ( 'NONE', #57394 ) ;
#99550=CIRCLE ( 'NONE', #43128, 0.09999999999999982514 ) ;
#99552=EDGE_LOOP ( 'NONE', ( #74460, #107648, #105377, #54158 ) ) ;
#99553=EDGE_LOOP ( 'NONE', ( #35045, #40404 ) ) ;
#99555=CARTESIAN_POINT ( 'NONE',  ( -4.800000000000024691, 2.500000000000000000, 4.676537180435972552 ) ) ;
#99556=ADVANCED_FACE ( 'NONE', ( #95385 ), #99931, .T. ) ;
#99557=CIRCLE ( 'NONE', #78723, 0.06509327318403741736 ) ;
#99558=CARTESIAN_POINT ( 'NONE',  ( -0.6000000000000383915, 12.50000000000000000, -3.918623584224389056 ) ) ;
#99560=CIRCLE ( 'NONE', #72371, 0.09999999999999982514 ) ;
#99561=EDGE_CURVE ( 'NONE', #31765, #126580, #100017, .T. ) ;
#99562=DIRECTION ( 'NONE',  ( 0.000000000000000000, 0.000000000000000000, 1.000000000000000000 ) ) ;
#99563=CARTESIAN_POINT ( 'NONE',  ( 4.799999999999937650, 2.500000000000000000, -0.2464101615137782308 ) ) ;
#99564=CARTESIAN_POINT ( 'NONE',  ( 11.24999999999990941, 2.500000000000000000, 7.088010851410848190 ) ) ;
#99565=FACE_OUTER_BOUND ( 'NONE', #75044, .T. ) ;
#99566=FACE_OUTER_BOUND ( 'NONE', #96393, .T. ) ;
#99567=EDGE_CURVE ( 'NONE', #96734, #99163, #33229, .T. ) ;
#99568=DIRECTION ( 'NONE',  ( -0.000000000000000000, -1.000000000000000000, -0.000000000000000000 ) ) ;
#99569=ORIENTED_EDGE ( 'NONE', *, *, #80188, .F. ) ;
#99570=CIRCLE ( 'NONE', #101621, 0.09999999999999982514 ) ;
#99571=ADVANCED_FACE ( 'NONE', ( #56715 ), #43698, .T. ) ;
#99572=ORIENTED_EDGE ( 'NONE', *, *, #32863, .F. ) ;
#99573=AXIS2_PLACEMENT_3D ( 'NONE', #69260, #107910, #67978 ) ;
#99574=CONICAL_SURFACE ( 'NONE', #34832, 0.1000000000000002554, 0.003490658503988666988 ) ;
#99575=ADVANCED_FACE ( 'NONE', ( #116936 ), #77029, .T. ) ;
#99576=CARTESIAN_POINT ( 'NONE',  ( 7.499999999999961808, 2.500000000000000000, 4.230127018922196669 ) ) ;
#99577=ORIENTED_EDGE ( 'NONE', *, *, #93619, .T. ) ;
#99578=ORIENTED_EDGE ( 'NONE', *, *, #38027, .T. ) ;
#99579=CARTESIAN_POINT ( 'NONE',  ( 6.649999999999927525, 12.50000000000000000, 2.230156782645134950 ) ) ;
#99580=EDGE_CURVE ( 'NONE', #125530, #50291, #36485, .T. ) ;
#99581=DIRECTION ( 'NONE',  ( 0.000000000000000000, 0.000000000000000000, 1.000000000000000000 ) ) ;
#99582=FACE_OUTER_BOUND ( 'NONE', #82626, .T. ) ;
#99583=LINE ( 'NONE', #79298, #7456 ) ;
#99584=CARTESIAN_POINT ( 'NONE',  ( -8.550000000000014921, 2.500000000000000000, -6.048780366869521252 ) ) ;
#99585=ORIENTED_EDGE ( 'NONE', *, *, #65676, .T. ) ;
#99586=VERTEX_POINT ( 'NONE', #115002 ) ;
#99587=CARTESIAN_POINT ( 'NONE',  ( 1.699999999999951994, 2.500000000000000000, -2.276824562219559311E-15 ) ) ;
#99590=ORIENTED_EDGE ( 'NONE', *, *, #43053, .T. ) ;
#99591=EDGE_CURVE ( 'NONE', #102898, #82416, #108415, .T. ) ;
#99592=ORIENTED_EDGE ( 'NONE', *, *, #68965, .F. ) ;
#99593=DIRECTION ( 'NONE',  ( 0.000000000000000000, -0.9999939076577903929, 0.003490651415223739937 ) ) ;
#99594=DIRECTION ( 'NONE',  ( 0.000000000000000000, 0.000000000000000000, -1.000000000000000000 ) ) ;
#99595=CIRCLE ( 'NONE', #49423, 0.1000000000000000472 ) ;
#99596=DIRECTION ( 'NONE',  ( 0.000000000000000000, 0.000000000000000000, 1.000000000000000000 ) ) ;
#99597=CIRCLE ( 'NONE', #103789, 0.06509327318403745899 ) ;
#99598=CARTESIAN_POINT ( 'NONE',  ( 10.19999999999991580, 2.500000000000000000, -0.3464101615137783474 ) ) ;
#99599=CARTESIAN_POINT ( 'NONE',  ( 87.50000000000002842, -0.7169905660283000248, 7.500000000000001776 ) ) ;
#99600=ORIENTED_EDGE ( 'NONE', *, *, #37626, .T. ) ;
#99601=CARTESIAN_POINT ( 'NONE',  ( 8.749999999999918288, 2.500000000000000000, 7.288010851410849256 ) ) ;
#99602=DIRECTION ( 'NONE',  ( -0.000000000000000000, -1.000000000000000000, -0.000000000000000000 ) ) ;
#99603=DIRECTION ( 'NONE',  ( 0.000000000000000000, 0.000000000000000000, 1.000000000000000000 ) ) ;
#99604=DIRECTION ( 'NONE',  ( -0.000000000000000000, -1.000000000000000000, -0.000000000000000000 ) ) ;
#99605=CIRCLE ( 'NONE', #62045, 0.06509327318403745899 ) ;
#99606=AXIS2_PLACEMENT_3D ( 'NONE', #44259, #43645, #114296 ) ;
#99607=CARTESIAN_POINT ( 'NONE',  ( 8.349999999999919709, 2.500000000000000000, 7.088010851410848190 ) ) ;
#99608=ORIENTED_EDGE ( 'NONE', *, *, #111622, .F. ) ;
#99609=ADVANCED_FACE ( 'NONE', ( #17443 ), #102165, .T. ) ;
#99610=ORIENTED_EDGE ( 'NONE', *, *, #112050, .T. ) ;
#99611=DIRECTION ( 'NONE',  ( 0.000000000000000000, 0.000000000000000000, 1.000000000000000000 ) ) ;
#99612=ORIENTED_EDGE ( 'NONE', *, *, #47914, .F. ) ;
#99613=VECTOR ( 'NONE', #44532, 1000.000000000000000 ) ;
#99614=CIRCLE ( 'NONE', #30672, 0.06509327318403745899 ) ;
#99615=CARTESIAN_POINT ( 'NONE',  ( 17.45053695044971676, -1.969637996572824568, 4.507340027902592361 ) ) ;
#99616=FACE_OUTER_BOUND ( 'NONE', #30859, .T. ) ;
#99617=AXIS2_PLACEMENT_3D ( 'NONE', #115805, #117719, #45793 ) ;
#99618=EDGE_LOOP ( 'NONE', ( #4036, #8979 ) ) ;
#99619=PLANE ( 'NONE',  #72412 ) ;
#99620=CARTESIAN_POINT ( 'NONE',  ( 11.84999999999990372, 12.50000000000000000, 2.446380397790835826 ) ) ;
#99621=ADVANCED_FACE ( 'NONE', ( #15517 ), #91699, .T. ) ;
#99622=FACE_OUTER_BOUND ( 'NONE', #84443, .T. ) ;
#99623=DIRECTION ( 'NONE',  ( -0.000000000000000000, -1.000000000000000000, -0.000000000000000000 ) ) ;
#99624=FACE_OUTER_BOUND ( 'NONE', #111237, .T. ) ;
#99625=EDGE_LOOP ( 'NONE', ( #126830, #58434 ) ) ;
#99626=DIRECTION ( 'NONE',  ( 0.000000000000000000, 0.000000000000000000, 1.000000000000000000 ) ) ;
#99627=DIRECTION ( 'NONE',  ( 0.000000000000000000, 1.000000000000000000, 0.000000000000000000 ) ) ;
#99628=DIRECTION ( 'NONE',  ( -0.000000000000000000, 1.000000000000000000, -0.000000000000000000 ) ) ;
#99629=VECTOR ( 'NONE', #85974, 1000.000000000000000 ) ;
#99630=VERTEX_POINT ( 'NONE', #5696 ) ;
#99631=CIRCLE ( 'NONE', #124677, 0.06509327318403745899 ) ;
#99632=CARTESIAN_POINT ( 'NONE',  ( 0.6499999999999561684, 12.50000000000000000, 2.511473670974873507 ) ) ;
#99633=CONICAL_SURFACE ( 'NONE', #42164, 0.1000000000000002554, 0.003490658503988666988 ) ;
#99634=ORIENTED_EDGE ( 'NONE', *, *, #110876, .F. ) ;
#99635=CARTESIAN_POINT ( 'NONE',  ( -7.700000000000016165, 2.500000000000000000, 0.3464101615137735735 ) ) ;
#99636=CARTESIAN_POINT ( 'NONE',  ( 11.64999999999990443, 12.50000000000000000, -7.253104124594891289 ) ) ;
#99637=VECTOR ( 'NONE', #128838, 1000.000000000000000 ) ;
#99638=FACE_OUTER_BOUND ( 'NONE', #69050, .T. ) ;
#99639=EDGE_LOOP ( 'NONE', ( #123651, #29776 ) ) ;
#99640=DIRECTION ( 'NONE',  ( 0.000000000000000000, 1.000000000000000000, 0.000000000000000000 ) ) ;
#99641=CIRCLE ( 'NONE', #101701, 0.06509327318403743123 ) ;
#99643=DIRECTION ( 'NONE',  ( -0.000000000000000000, 1.000000000000000000, -0.000000000000000000 ) ) ;
#99644=VERTEX_POINT ( 'NONE', #26643 ) ;
#99645=CARTESIAN_POINT ( 'NONE',  ( 8.549999999999922551, 2.500000000000000000, 2.511473670974873507 ) ) ;
#99646=VERTEX_POINT ( 'NONE', #66553 ) ;
#99648=EDGE_CURVE ( 'NONE', #6400, #67035, #35818, .T. ) ;
#99649=CIRCLE ( 'NONE', #126838, 0.06509327318403745899 ) ;
#99650=AXIS2_PLACEMENT_3D ( 'NONE', #66669, #44464, #45121 ) ;
#99651=EDGE_LOOP ( 'NONE', ( #15500, #56404, #97707, #86083 ) ) ;
#99652=CARTESIAN_POINT ( 'NONE',  ( -4.150000000000025224, 2.500000000000000000, 5.902370205355745192 ) ) ;
#99653=CARTESIAN_POINT ( 'NONE',  ( 14.93814514904464197, 2.500000000000000000, -6.173787961026619087 ) ) ;
#99654=EDGE_CURVE ( 'NONE', #46914, #92524, #31078, .T. ) ;
#99655=EDGE_LOOP ( 'NONE', ( #111406, #27205, #96949, #31996 ) ) ;
#99656=EDGE_CURVE ( 'NONE', #26594, #19417, #56091, .T. ) ;
#99657=VERTEX_POINT ( 'NONE', #122052 ) ;
#99659=EDGE_CURVE ( 'NONE', #27686, #6619, #123963, .T. ) ;
#99660=DIRECTION ( 'NONE',  ( -0.000000000000000000, -1.000000000000000000, -0.000000000000000000 ) ) ;
#99661=DIRECTION ( 'NONE',  ( 0.000000000000000000, 0.000000000000000000, 1.000000000000000000 ) ) ;
#99662=ORIENTED_EDGE ( 'NONE', *, *, #12211, .F. ) ;
#99663=DIRECTION ( 'NONE',  ( -4.274815082592931898E-19, -0.9999939076577903929, -0.003490651415223739937 ) ) ;
#99664=DIRECTION ( 'NONE',  ( -0.000000000000000000, 1.000000000000000000, -0.000000000000000000 ) ) ;
#99665=ADVANCED_FACE ( 'NONE', ( #23186 ), #42869, .T. ) ;
#99666=FACE_OUTER_BOUND ( 'NONE', #40135, .T. ) ;
#99667=EDGE_CURVE ( 'NONE', #3622, #20697, #102409, .T. ) ;
#99668=CARTESIAN_POINT ( 'NONE',  ( 3.099999999999944134, 2.500000000000000000, 4.776537180435972196 ) ) ;
#99669=CARTESIAN_POINT ( 'NONE',  ( -6.250000000000019540, 12.50000000000000000, -2.922977105672691422 ) ) ;
#99670=CARTESIAN_POINT ( 'NONE',  ( 4.549999999999937650, 12.50000000000000000, 2.230156782645134950 ) ) ;
#99671=CARTESIAN_POINT ( 'NONE',  ( -1.050000000000038680, 2.500000000000000000, 6.741600689897071952 ) ) ;
#99672=CIRCLE ( 'NONE', #28663, 0.06509327318403745899 ) ;
#99673=ADVANCED_FACE ( 'NONE', ( #42200 ), #20595, .T. ) ;
#99674=EDGE_CURVE ( 'NONE', #67302, #98804, #104953, .T. ) ;
#99675=EDGE_CURVE ( 'NONE', #112457, #65686, #63115, .T. ) ;
#99676=ORIENTED_EDGE ( 'NONE', *, *, #67994, .T. ) ;
#99677=ORIENTED_EDGE ( 'NONE', *, *, #72956, .F. ) ;
#99678=ORIENTED_EDGE ( 'NONE', *, *, #13776, .F. ) ;
#99679=ORIENTED_EDGE ( 'NONE', *, *, #67993, .F. ) ;
#99680=CARTESIAN_POINT ( 'NONE',  ( -7.050000000000013145, 2.500000000000000000, 2.165063509461097713 ) ) ;
#99681=FACE_OUTER_BOUND ( 'NONE', #52623, .T. ) ;
#99682=DIRECTION ( 'NONE',  ( 0.000000000000000000, 0.000000000000000000, -1.000000000000000000 ) ) ;
#99683=ORIENTED_EDGE ( 'NONE', *, *, #50647, .F. ) ;
#99684=FACE_BOUND ( 'NONE', #91202, .T. ) ;
#99685=ORIENTED_EDGE ( 'NONE', *, *, #15603, .F. ) ;
#99686=ADVANCED_FACE ( 'NONE', ( #25122 ), #127217, .T. ) ;
#99687=DIRECTION ( 'NONE',  ( 0.000000000000000000, 0.000000000000000000, 1.000000000000000000 ) ) ;
#99688=DIRECTION ( 'NONE',  ( 0.000000000000000000, 0.000000000000000000, 1.000000000000000000 ) ) ;
#99689=DIRECTION ( 'NONE',  ( 0.000000000000000000, 0.000000000000000000, -1.000000000000000000 ) ) ;
#99690=VECTOR ( 'NONE', #75220, 1000.000000000000000 ) ;
#99691=DIRECTION ( 'NONE',  ( -0.000000000000000000, -1.000000000000000000, -0.000000000000000000 ) ) ;
#99692=CIRCLE ( 'NONE', #7717, 0.1000000000000002554 ) ;
#99693=DIRECTION ( 'NONE',  ( 0.000000000000000000, 0.000000000000000000, -1.000000000000000000 ) ) ;
#99694=DIRECTION ( 'NONE',  ( 0.000000000000000000, 0.000000000000000000, 1.000000000000000000 ) ) ;
#99695=CARTESIAN_POINT ( 'NONE',  ( 0.8499999999999553468, 2.500000000000000000, 1.472243186433545459 ) ) ;
#99696=CARTESIAN_POINT ( 'NONE',  ( -1.450000000000035039, 12.50000000000000000, -2.511473670974877948 ) ) ;
#99697=DIRECTION ( 'NONE',  ( 0.000000000000000000, 1.000000000000000000, 0.000000000000000000 ) ) ;
#99698=VECTOR ( 'NONE', #118440, 1000.000000000000000 ) ;
#99699=CIRCLE ( 'NONE', #3539, 0.06509327318403745899 ) ;
#99700=EDGE_LOOP ( 'NONE', ( #40569, #85362 ) ) ;
#99701=VERTEX_POINT ( 'NONE', #23852 ) ;
#99702=ORIENTED_EDGE ( 'NONE', *, *, #71387, .F. ) ;
#99703=VERTEX_POINT ( 'NONE', #14640 ) ;
#99704=LINE ( 'NONE', #119317, #87335 ) ;
#99705=DIRECTION ( 'NONE',  ( -4.274815082592931898E-19, -0.9999939076577903929, -0.003490651415223739937 ) ) ;
#99706=EDGE_LOOP ( 'NONE', ( #81815, #87001, #17106, #54058 ) ) ;
#99707=EDGE_LOOP ( 'NONE', ( #51238, #127526 ) ) ;
#99708=ORIENTED_EDGE ( 'NONE', *, *, #1132, .T. ) ;
#99709=DIRECTION ( 'NONE',  ( -4.274815082592931898E-19, -0.9999939076577903929, -0.003490651415223739937 ) ) ;
#99710=CIRCLE ( 'NONE', #80924, 0.1000000000000000472 ) ;
#99711=AXIS2_PLACEMENT_3D ( 'NONE', #125262, #46065, #54569 ) ;
#99712=DIRECTION ( 'NONE',  ( 0.000000000000000000, 0.000000000000000000, 1.000000000000000000 ) ) ;
#99713=CARTESIAN_POINT ( 'NONE',  ( -1.850000000000033840, 2.500000000000000000, 1.718653347947321386 ) ) ;
#99714=DIRECTION ( 'NONE',  ( 0.000000000000000000, 1.000000000000000000, 0.000000000000000000 ) ) ;
#99715=DIRECTION ( 'NONE',  ( 0.000000000000000000, 0.000000000000000000, 1.000000000000000000 ) ) ;
#99716=CARTESIAN_POINT ( 'NONE',  ( 2.500000000000001776, 2.021986658763283096, 9.892226903609811828 ) ) ;
#99717=CARTESIAN_POINT ( 'NONE',  ( 6.449999999999931788, 2.500000000000000000, -6.148780366869526226 ) ) ;
#99718=ORIENTED_EDGE ( 'NONE', *, *, #38361, .F. ) ;
#99719=DIRECTION ( 'NONE',  ( 0.000000000000000000, 1.000000000000000000, 0.000000000000000000 ) ) ;
#99720=VERTEX_POINT ( 'NONE', #55243 ) ;
#99721=EDGE_CURVE ( 'NONE', #3084, #46462, #3864, .T. ) ;
#99722=VERTEX_POINT ( 'NONE', #2248 ) ;
#99723=ORIENTED_EDGE ( 'NONE', *, *, #116495, .T. ) ;
#99724=EDGE_CURVE ( 'NONE', #69063, #86941, #16463, .T. ) ;
#99725=DIRECTION ( 'NONE',  ( -0.000000000000000000, -1.000000000000000000, -0.000000000000000000 ) ) ;
#99726=ORIENTED_EDGE ( 'NONE', *, *, #19611, .F. ) ;
#99727=ORIENTED_EDGE ( 'NONE', *, *, #90389, .F. ) ;
#99728=AXIS2_PLACEMENT_3D ( 'NONE', #11780, #51724, #91636 ) ;
#99729=AXIS2_PLACEMENT_3D ( 'NONE', #38707, #77310, #118516 ) ;
#99730=DIRECTION ( 'NONE',  ( 0.000000000000000000, 0.000000000000000000, 1.000000000000000000 ) ) ;
#99731=EDGE_CURVE ( 'NONE', #72821, #32401, #51994, .T. ) ;
#99732=DIRECTION ( 'NONE',  ( -4.274815082592931898E-19, -0.9999939076577903929, -0.003490651415223739937 ) ) ;
#99733=CARTESIAN_POINT ( 'NONE',  ( 2.299999999999948752, 12.50000000000000000, -3.983716857408426293 ) ) ;
#99734=AXIS2_PLACEMENT_3D ( 'NONE', #42838, #12047, #2887 ) ;
#99735=CARTESIAN_POINT ( 'NONE',  ( 9.599999999999914380, 2.500000000000000000, 4.922947341949748257 ) ) ;
#99736=DIRECTION ( 'NONE',  ( 0.000000000000000000, -0.9999939076577903929, 0.003490651415223739937 ) ) ;
#99737=AXIS2_PLACEMENT_3D ( 'NONE', #44942, #22737, #103208 ) ;
#99738=ORIENTED_EDGE ( 'NONE', *, *, #34591, .T. ) ;
#99739=DIRECTION ( 'NONE',  ( -0.000000000000000000, 1.000000000000000000, -0.000000000000000000 ) ) ;
#99740=CIRCLE ( 'NONE', #39211, 0.06509327318403741736 ) ;
#99742=AXIS2_PLACEMENT_3D ( 'NONE', #51169, #110706, #80626 ) ;
#99743=LINE ( 'NONE', #78168, #4493 ) ;
#99744=ORIENTED_EDGE ( 'NONE', *, *, #58323, .F. ) ;
#99746=DIRECTION ( 'NONE',  ( 0.000000000000000000, 0.000000000000000000, 1.000000000000000000 ) ) ;
#99747=ORIENTED_EDGE ( 'NONE', *, *, #5371, .F. ) ;
#99748=FACE_OUTER_BOUND ( 'NONE', #105652, .T. ) ;
#99749=CIRCLE ( 'NONE', #103851, 0.06509327318403745899 ) ;
#99750=CARTESIAN_POINT ( 'NONE',  ( -11.64999999999999680, 2.500000000000000000, -2.165063509461097713 ) ) ;
#99751=EDGE_LOOP ( 'NONE', ( #102745, #91383, #44301, #72521 ) ) ;
#99752=VECTOR ( 'NONE', #82169, 1000.000000000000000 ) ;
#99753=VECTOR ( 'NONE', #73122, 1000.000000000000000 ) ;
#99754=DIRECTION ( 'NONE',  ( 0.000000000000000000, 0.000000000000000000, -1.000000000000000000 ) ) ;
#99756=ORIENTED_EDGE ( 'NONE', *, *, #32016, .T. ) ;
#99757=DIRECTION ( 'NONE',  ( 0.000000000000000000, 0.000000000000000000, 1.000000000000000000 ) ) ;
#99758=DIRECTION ( 'NONE',  ( 0.000000000000000000, -0.9999939076577903929, 0.003490651415223739937 ) ) ;
#99759=CARTESIAN_POINT ( 'NONE',  ( -15.19999999999998330, 12.50000000000000000, 0.2813168883297384459 ) ) ;
#99760=CARTESIAN_POINT ( 'NONE',  ( -5.200000000000025935, 12.50000000000000000, -3.983716857408426293 ) ) ;
#99761=DIRECTION ( 'NONE',  ( 0.000000000000000000, 0.000000000000000000, 1.000000000000000000 ) ) ;
#99762=VERTEX_POINT ( 'NONE', #103036 ) ;
#99763=CARTESIAN_POINT ( 'NONE',  ( -1.250000000000037526, 2.500000000000000000, -1.472243186433550122 ) ) ;
#99764=CIRCLE ( 'NONE', #97605, 0.09999999999999982514 ) ;
#99765=ORIENTED_EDGE ( 'NONE', *, *, #93907, .T. ) ;
#99766=DIRECTION ( 'NONE',  ( -0.000000000000000000, 1.000000000000000000, -0.000000000000000000 ) ) ;
#99767=DIRECTION ( 'NONE',  ( 0.000000000000000000, 0.000000000000000000, 1.000000000000000000 ) ) ;
#99770=DIRECTION ( 'NONE',  ( 0.000000000000000000, 1.000000000000000000, 0.000000000000000000 ) ) ;
#99771=DIRECTION ( 'NONE',  ( 0.000000000000000000, -0.000000000000000000, 1.000000000000000000 ) ) ;
#99772=EDGE_CURVE ( 'NONE', #40007, #14402, #85432, .T. ) ;
#99773=CARTESIAN_POINT ( 'NONE',  ( -8.750000000000008882, 2.500000000000000000, -2.857883832488653741 ) ) ;
#99775=ORIENTED_EDGE ( 'NONE', *, *, #29746, .T. ) ;
#99776=FACE_OUTER_BOUND ( 'NONE', #94374, .T. ) ;
#99777=CONICAL_SURFACE ( 'NONE', #72681, 0.09999999999999982514, 0.003490658503988666988 ) ;
#99778=PLANE ( 'NONE',  #45140 ) ;
#99779=CARTESIAN_POINT ( 'NONE',  ( -8.150000000000012790, 12.50000000000000000, 2.511473670974873507 ) ) ;
#99780=EDGE_CURVE ( 'NONE', #34236, #109647, #1795, .T. ) ;
#99781=ORIENTED_EDGE ( 'NONE', *, *, #78727, .T. ) ;
#99783=CIRCLE ( 'NONE', #124826, 0.06509327318403745899 ) ;
#99784=LINE ( 'NONE', #79501, #88720 ) ;
#99785=AXIS2_PLACEMENT_3D ( 'NONE', #46570, #75383, #25007 ) ;
#99786=ORIENTED_EDGE ( 'NONE', *, *, #66425, .F. ) ;
#99788=CARTESIAN_POINT ( 'NONE',  ( 2.949999999999945111, 2.500000000000000000, 2.165063509461097713 ) ) ;
#99789=EDGE_LOOP ( 'NONE', ( #34571, #52750, #9779, #79704 ) ) ;
#99790=FACE_OUTER_BOUND ( 'NONE', #39899, .T. ) ;
#99792=AXIS2_PLACEMENT_3D ( 'NONE', #126651, #78201, #127934 ) ;
#99793=AXIS2_PLACEMENT_3D ( 'NONE', #1915, #32702, #22230 ) ;
#99794=ORIENTED_EDGE ( 'NONE', *, *, #12659, .F. ) ;
#99795=DIRECTION ( 'NONE',  ( 0.000000000000000000, 0.000000000000000000, -1.000000000000000000 ) ) ;
#99796=ADVANCED_FACE ( 'NONE', ( #14002 ), #93871, .T. ) ;
#99797=DIRECTION ( 'NONE',  ( 0.000000000000000000, 0.000000000000000000, 1.000000000000000000 ) ) ;
#99798=DIRECTION ( 'NONE',  ( -0.000000000000000000, 1.000000000000000000, -0.000000000000000000 ) ) ;
#99799=ORIENTED_EDGE ( 'NONE', *, *, #51542, .F. ) ;
#99800=ADVANCED_FACE ( 'NONE', ( #104333 ), #79192, .T. ) ;
#99801=AXIS2_PLACEMENT_3D ( 'NONE', #115423, #25779, #4189 ) ;
#99803=ORIENTED_EDGE ( 'NONE', *, *, #41924, .F. ) ;
#99804=CONICAL_SURFACE ( 'NONE', #70549, 0.1000000000000000472, 0.003490658503988666988 ) ;
#99805=DIRECTION ( 'NONE',  ( -0.000000000000000000, -1.000000000000000000, -0.000000000000000000 ) ) ;
#99806=DIRECTION ( 'NONE',  ( -0.000000000000000000, 1.000000000000000000, -0.000000000000000000 ) ) ;
#99807=CARTESIAN_POINT ( 'NONE',  ( 11.64999999999990798, 2.500000000000000000, 7.188010851410848723 ) ) ;
#99808=EDGE_CURVE ( 'NONE', #43427, #122964, #62467, .T. ) ;
#99809=EDGE_CURVE ( 'NONE', #88819, #99762, #79768, .T. ) ;
#99810=FACE_BOUND ( 'NONE', #82115, .T. ) ;
#99811=ORIENTED_EDGE ( 'NONE', *, *, #59636, .F. ) ;
#99812=ADVANCED_FACE ( 'NONE', ( #90876 ), #30040, .T. ) ;
#99813=CIRCLE ( 'NONE', #30874, 0.1000000000000002554 ) ;
#99814=EDGE_CURVE ( 'NONE', #128968, #103425, #9742, .T. ) ;
#99816=DIRECTION ( 'NONE',  ( 0.000000000000000000, 1.000000000000000000, 0.000000000000000000 ) ) ;
#99817=VECTOR ( 'NONE', #80545, 1000.000000000000000 ) ;
#99818=ORIENTED_EDGE ( 'NONE', *, *, #33380, .T. ) ;
#99819=DIRECTION ( 'NONE',  ( 0.000000000000000000, 0.000000000000000000, 1.000000000000000000 ) ) ;
#99820=CARTESIAN_POINT ( 'NONE',  ( 3.949999999999942446, 2.500000000000000000, -6.841600689897078702 ) ) ;
#99821=CIRCLE ( 'NONE', #124942, 0.06509327318403745899 ) ;
#99822=ADVANCED_FACE ( 'NONE', ( #30691 ), #129383, .T. ) ;
#99823=DIRECTION ( 'NONE',  ( 0.000000000000000000, 1.000000000000000000, 0.000000000000000000 ) ) ;
#99824=PLANE ( 'NONE',  #48663 ) ;
#99825=DIRECTION ( 'NONE',  ( 1.000000000000000000, 0.000000000000000000, 0.000000000000000000 ) ) ;
#99826=EDGE_CURVE ( 'NONE', #49458, #51199, #22806, .T. ) ;
#99827=CARTESIAN_POINT ( 'NONE',  ( 8.749999999999920064, 12.50000000000000000, 5.867463478539781896 ) ) ;
#99828=AXIS2_PLACEMENT_3D ( 'NONE', #78925, #69075, #39654 ) ;
#99829=DIRECTION ( 'NONE',  ( 0.000000000000000000, 1.000000000000000000, 0.000000000000000000 ) ) ;
#99830=CIRCLE ( 'NONE', #108225, 0.06509327318403745899 ) ;
#99831=CIRCLE ( 'NONE', #22484, 9.000000000000001776 ) ;
#99832=CONICAL_SURFACE ( 'NONE', #28821, 0.1000000000000002554, 0.003490658503988666988 ) ;
#99833=EDGE_CURVE ( 'NONE', #64891, #103728, #89645, .T. ) ;
#99834=VERTEX_POINT ( 'NONE', #20210 ) ;
#99835=ORIENTED_EDGE ( 'NONE', *, *, #60469, .T. ) ;
#99836=ORIENTED_EDGE ( 'NONE', *, *, #35919, .F. ) ;
#99837=ORIENTED_EDGE ( 'NONE', *, *, #59365, .T. ) ;
#99838=DIRECTION ( 'NONE',  ( 0.000000000000000000, 0.000000000000000000, -1.000000000000000000 ) ) ;
#99839=DIRECTION ( 'NONE',  ( -0.000000000000000000, 1.000000000000000000, -0.000000000000000000 ) ) ;
#99840=EDGE_LOOP ( 'NONE', ( #68063, #65584, #86734, #104538 ) ) ;
#99841=EDGE_CURVE ( 'NONE', #70779, #122261, #60423, .T. ) ;
#99842=FACE_BOUND ( 'NONE', #25983, .T. ) ;
#99843=EDGE_CURVE ( 'NONE', #64309, #127944, #37429, .T. ) ;
#99844=CARTESIAN_POINT ( 'NONE',  ( -1.650000000000035660, 12.50000000000000000, 2.922977105672686982 ) ) ;
#99845=CONICAL_SURFACE ( 'NONE', #89458, 0.1000000000000002554, 0.003490658503988666988 ) ;
#99846=DIRECTION ( 'NONE',  ( -0.000000000000000000, -1.000000000000000000, -0.000000000000000000 ) ) ;
#99847=DIRECTION ( 'NONE',  ( 0.000000000000000000, -0.000000000000000000, 1.000000000000000000 ) ) ;
#99848=FACE_OUTER_BOUND ( 'NONE', #20862, .T. ) ;
#99849=CARTESIAN_POINT ( 'NONE',  ( -6.650000000000014566, 2.500000000000000000, 5.702370205355745014 ) ) ;
#99850=DIRECTION ( 'NONE',  ( 0.000000000000000000, 0.000000000000000000, -1.000000000000000000 ) ) ;
#99851=ORIENTED_EDGE ( 'NONE', *, *, #97270, .T. ) ;
#99852=VERTEX_POINT ( 'NONE', #41804 ) ;
#99853=EDGE_LOOP ( 'NONE', ( #52906, #72653, #36275, #23453 ) ) ;
#99854=ORIENTED_EDGE ( 'NONE', *, *, #22832, .T. ) ;
#99855=EDGE_LOOP ( 'NONE', ( #103659, #114750, #59729, #74584 ) ) ;
#99856=ORIENTED_EDGE ( 'NONE', *, *, #36573, .F. ) ;
#99857=DIRECTION ( 'NONE',  ( 0.000000000000000000, 0.000000000000000000, 1.000000000000000000 ) ) ;
#99858=CARTESIAN_POINT ( 'NONE',  ( 6.649999999999927525, 2.500000000000000000, 2.165063509461097713 ) ) ;
#99859=ORIENTED_EDGE ( 'NONE', *, *, #19538, .F. ) ;
#99860=AXIS2_PLACEMENT_3D ( 'NONE', #117298, #38134, #27643 ) ;
#99861=CARTESIAN_POINT ( 'NONE',  ( -4.400000000000025224, 12.50000000000000000, 4.676537180435972552 ) ) ;
#99862=CARTESIAN_POINT ( 'NONE',  ( -0.8500000000000386136, 2.500000000000000000, 2.857883832488649301 ) ) ;
#99863=CARTESIAN_POINT ( 'NONE',  ( 4.149999999999938183, 12.50000000000000000, 2.165063509461097713 ) ) ;
#99865=LINE ( 'NONE', #10190, #50037 ) ;
#99866=DIRECTION ( 'NONE',  ( 0.000000000000000000, 0.000000000000000000, 1.000000000000000000 ) ) ;
#99867=DIRECTION ( 'NONE',  ( -0.000000000000000000, -1.000000000000000000, -0.000000000000000000 ) ) ;
#99868=ORIENTED_EDGE ( 'NONE', *, *, #58141, .F. ) ;
#99869=DIRECTION ( 'NONE',  ( -0.000000000000000000, -1.000000000000000000, -0.000000000000000000 ) ) ;
#99870=AXIS2_PLACEMENT_3D ( 'NONE', #23380, #63314, #103249 ) ;
#99871=EDGE_LOOP ( 'NONE', ( #70821, #30613, #99425, #127700 ) ) ;
#99872=EDGE_CURVE ( 'NONE', #82187, #105036, #91791, .T. ) ;
#99873=VECTOR ( 'NONE', #72098, 1000.000000000000000 ) ;
#99874=VERTEX_POINT ( 'NONE', #550 ) ;
#99875=FACE_OUTER_BOUND ( 'NONE', #121160, .T. ) ;
#99876=EDGE_CURVE ( 'NONE', #56688, #105502, #114760, .T. ) ;
#99877=CARTESIAN_POINT ( 'NONE',  ( 12.69999999999990337, 2.500000000000000000, 3.983716857408420076 ) ) ;
#99878=CARTESIAN_POINT ( 'NONE',  ( -0.2000000000000408673, 12.50000000000000000, -3.983716857408426293 ) ) ;
#99879=EDGE_LOOP ( 'NONE', ( #56537, #14486, #16010, #13041 ) ) ;
#99881=EDGE_LOOP ( 'NONE', ( #104531, #57932 ) ) ;
#99882=DIRECTION ( 'NONE',  ( 0.000000000000000000, 0.000000000000000000, 1.000000000000000000 ) ) ;
#99883=VECTOR ( 'NONE', #27565, 1000.000000000000000 ) ;
#99884=AXIS2_PLACEMENT_3D ( 'NONE', #78128, #19852, #106917 ) ;
#99885=CARTESIAN_POINT ( 'NONE',  ( 6.899999999999928413, 2.500000000000000000, -4.676537180435977881 ) ) ;
#99886=DIRECTION ( 'NONE',  ( 0.000000000000000000, 1.000000000000000000, 0.000000000000000000 ) ) ;
#99887=DIRECTION ( 'NONE',  ( 0.000000000000000000, 0.000000000000000000, 1.000000000000000000 ) ) ;
#99888=VERTEX_POINT ( 'NONE', #40515 ) ;
#99889=CARTESIAN_POINT ( 'NONE',  ( 3.149999999999944400, 12.50000000000000000, 2.576566944158910744 ) ) ;
#99890=ORIENTED_EDGE ( 'NONE', *, *, #94648, .T. ) ;
#99891=CARTESIAN_POINT ( 'NONE',  ( -4.119968255444916849E-14, 2.500000000000000000, 3.737306695894644371 ) ) ;
#99892=ORIENTED_EDGE ( 'NONE', *, *, #128001, .T. ) ;
#99893=FACE_OUTER_BOUND ( 'NONE', #70077, .T. ) ;
#99894=FACE_OUTER_BOUND ( 'NONE', #90832, .T. ) ;
#99895=CARTESIAN_POINT ( 'NONE',  ( 6.649999999999931966, 12.50000000000000000, -5.802370205355749988 ) ) ;
#99896=AXIS2_PLACEMENT_3D ( 'NONE', #71567, #11362, #70292 ) ;
#99897=CARTESIAN_POINT ( 'NONE',  ( 8.349999999999923261, 12.50000000000000000, -5.737276932171712751 ) ) ;
#99898=EDGE_LOOP ( 'NONE', ( #60851, #69717, #43806, #6446 ) ) ;
#99899=CARTESIAN_POINT ( 'NONE',  ( -11.64999999999999680, 12.50000000000000000, 6.560283801567334372 ) ) ;
#99900=CONICAL_SURFACE ( 'NONE', #120821, 0.1000000000000002554, 0.003490658503988666988 ) ;
#99901=AXIS2_PLACEMENT_3D ( 'NONE', #118690, #30339, #193 ) ;
#99902=FACE_OUTER_BOUND ( 'NONE', #19190, .T. ) ;
#99903=EDGE_LOOP ( 'NONE', ( #27400, #28124 ) ) ;
#99904=ORIENTED_EDGE ( 'NONE', *, *, #99337, .F. ) ;
#99905=DIRECTION ( 'NONE',  ( -0.000000000000000000, -1.000000000000000000, -0.000000000000000000 ) ) ;
#99906=CARTESIAN_POINT ( 'NONE',  ( 8.549999999999918998, 2.500000000000000000, 6.741600689897071952 ) ) ;
#99907=DIRECTION ( 'NONE',  ( -0.000000000000000000, -1.000000000000000000, -0.000000000000000000 ) ) ;
#99908=CIRCLE ( 'NONE', #30968, 0.1000000000000002554 ) ;
#99909=FACE_OUTER_BOUND ( 'NONE', #461, .T. ) ;
#99910=VECTOR ( 'NONE', #88423, 1000.000000000000000 ) ;
#99911=DIRECTION ( 'NONE',  ( 0.000000000000000000, -0.000000000000000000, 1.000000000000000000 ) ) ;
#99912=EDGE_CURVE ( 'NONE', #56997, #123277, #87572, .T. ) ;
#99913=AXIS2_PLACEMENT_3D ( 'NONE', #83981, #94448, #5424 ) ;
#99914=CARTESIAN_POINT ( 'NONE',  ( 2.499999999999948930, 12.50000000000000000, -0.6928203230275541413 ) ) ;
#99915=PLANE ( 'NONE',  #120177 ) ;
#99917=CIRCLE ( 'NONE', #43489, 0.1000000000000002554 ) ;
#99918=ADVANCED_FACE ( 'NONE', ( #80427 ), #45828, .T. ) ;
#99919=VECTOR ( 'NONE', #14905, 1000.000000000000000 ) ;
#99920=EDGE_LOOP ( 'NONE', ( #126469, #112052 ) ) ;
#99921=CARTESIAN_POINT ( 'NONE',  ( 13.14999999999990088, 2.500000000000000000, 1.818653347947321475 ) ) ;
#99923=CIRCLE ( 'NONE', #7871, 0.06509327318403745899 ) ;
#99924=DIRECTION ( 'NONE',  ( 0.000000000000000000, 0.000000000000000000, -1.000000000000000000 ) ) ;
#99925=CARTESIAN_POINT ( 'NONE',  ( -6.650000000000019007, 12.50000000000000000, -1.472243186433550122 ) ) ;
#99926=EDGE_CURVE ( 'NONE', #17094, #34777, #50972, .T. ) ;
#99927=CARTESIAN_POINT ( 'NONE',  ( -11.44999999999999929, 2.500000000000000000, -1.918653347947322230 ) ) ;
#99928=FACE_OUTER_BOUND ( 'NONE', #97652, .T. ) ;
#99929=VERTEX_POINT ( 'NONE', #71230 ) ;
#99930=CARTESIAN_POINT ( 'NONE',  ( -7.900000000000014566, 12.50000000000000000, -4.265033745738164406 ) ) ;
#99931=CONICAL_SURFACE ( 'NONE', #47788, 0.1000000000000002554, 0.003490658503988666988 ) ;
#99932=AXIS2_PLACEMENT_3D ( 'NONE', #339, #79571, #9541 ) ;
#99933=PLANE ( 'NONE',  #7275 ) ;
#99934=CARTESIAN_POINT ( 'NONE',  ( 8.749999999999957367, 12.50000000000000000, 2.165063509461097713 ) ) ;
#99935=VERTEX_POINT ( 'NONE', #111819 ) ;
#99936=EDGE_CURVE ( 'NONE', #116685, #94318, #31172, .T. ) ;
#99937=ORIENTED_EDGE ( 'NONE', *, *, #3504, .T. ) ;
#99938=CARTESIAN_POINT ( 'NONE',  ( 7.099999999999927702, 2.500000000000000000, -3.637306695894650055 ) ) ;
#99940=ORIENTED_EDGE ( 'NONE', *, *, #82505, .T. ) ;
#99941=FACE_OUTER_BOUND ( 'NONE', #18693, .T. ) ;
#99942=DIRECTION ( 'NONE',  ( 0.000000000000000000, 0.000000000000000000, 1.000000000000000000 ) ) ;
#99943=DIRECTION ( 'NONE',  ( -0.000000000000000000, 1.000000000000000000, -0.000000000000000000 ) ) ;
#99944=CARTESIAN_POINT ( 'NONE',  ( -3.750000000000025757, 2.500000000000000000, 1.372243186433545370 ) ) ;
#99945=VERTEX_POINT ( 'NONE', #2477 ) ;
#99946=AXIS2_PLACEMENT_3D ( 'NONE', #19682, #11782, #59630 ) ;
#99949=DIRECTION ( 'NONE',  ( 0.000000000000000000, -0.000000000000000000, 1.000000000000000000 ) ) ;
#99950=CIRCLE ( 'NONE', #60260, 0.06509327318403745899 ) ;
#99951=DIRECTION ( 'NONE',  ( 0.000000000000000000, 1.000000000000000000, 0.000000000000000000 ) ) ;
#99952=DIRECTION ( 'NONE',  ( 0.000000000000000000, 0.000000000000000000, 1.000000000000000000 ) ) ;
#99953=ORIENTED_EDGE ( 'NONE', *, *, #18657, .F. ) ;
#99954=CIRCLE ( 'NONE', #3806, 0.06509327318403745899 ) ;
#99955=EDGE_CURVE ( 'NONE', #107304, #46456, #116904, .T. ) ;
#99956=CIRCLE ( 'NONE', #106306, 0.06509327318403745899 ) ;
#99958=EDGE_LOOP ( 'NONE', ( #115876, #72176, #36012, #48582 ) ) ;
#99959=EDGE_LOOP ( 'NONE', ( #83119, #47212, #78885, #115391 ) ) ;
#99960=VERTEX_POINT ( 'NONE', #72542 ) ;
#99961=DIRECTION ( 'NONE',  ( 0.000000000000000000, 0.000000000000000000, 1.000000000000000000 ) ) ;
#99962=CARTESIAN_POINT ( 'NONE',  ( 12.65326442612249735, 2.499999999999999112, 8.428886917614240915 ) ) ;
#99963=DIRECTION ( 'NONE',  ( -0.000000000000000000, 1.000000000000000000, -0.000000000000000000 ) ) ;
#99964=ADVANCED_FACE ( 'NONE', ( #105202 ), #41646, .T. ) ;
#99965=FACE_BOUND ( 'NONE', #103087, .T. ) ;
#99966=CARTESIAN_POINT ( 'NONE',  ( -2.500000000000032419, 2.500000000000000000, 0.7928203230275495672 ) ) ;
#99968=CONICAL_SURFACE ( 'NONE', #110421, 0.1000000000000000472, 0.003490658503988666988 ) ;
#99969=EDGE_CURVE ( 'NONE', #39409, #45762, #22858, .T. ) ;
#99970=DIRECTION ( 'NONE',  ( -0.000000000000000000, -1.000000000000000000, -0.000000000000000000 ) ) ;
#99971=CARTESIAN_POINT ( 'NONE',  ( 8.749999999999918288, 2.500000000000000000, -1.572243186433550211 ) ) ;
#99972=CIRCLE ( 'NONE', #35143, 0.06509327318403745899 ) ;
#99973=EDGE_CURVE ( 'NONE', #41348, #115380, #3952, .T. ) ;
#99974=CARTESIAN_POINT ( 'NONE',  ( -4.350000000000027178, 12.50000000000000000, -6.841600689897077814 ) ) ;
#99975=EDGE_CURVE ( 'NONE', #27857, #113935, #68806, .T. ) ;
#99976=DIRECTION ( 'NONE',  ( 0.000000000000000000, 1.000000000000000000, 0.000000000000000000 ) ) ;
#99977=EDGE_CURVE ( 'NONE', #35495, #99852, #127306, .T. ) ;
#99978=CARTESIAN_POINT ( 'NONE',  ( 4.799999999999939426, 2.500000000000000000, -4.676537180435977881 ) ) ;
#99979=EDGE_CURVE ( 'NONE', #93665, #37844, #12363, .T. ) ;
#99980=VECTOR ( 'NONE', #64734, 1000.000000000000000 ) ;
#99981=CARTESIAN_POINT ( 'NONE',  ( -6.700000000000019718, 2.500000000000000000, -4.330127018922201643 ) ) ;
#99982=EDGE_CURVE ( 'NONE', #79044, #26093, #60510, .T. ) ;
#99983=VERTEX_POINT ( 'NONE', #63354 ) ;
#99984=VERTEX_POINT ( 'NONE', #93456 ) ;
#99985=ORIENTED_EDGE ( 'NONE', *, *, #49763, .F. ) ;
#99986=ORIENTED_EDGE ( 'NONE', *, *, #52681, .T. ) ;
#99987=CONICAL_SURFACE ( 'NONE', #98001, 0.09999999999999982514, 0.003490658503988666988 ) ;
#99988=CARTESIAN_POINT ( 'NONE',  ( 9.549999999999918998, 2.500000000000000000, -6.395190528383301931 ) ) ;
#99989=LINE ( 'NONE', #18833, #103028 ) ;
#99990=FACE_BOUND ( 'NONE', #83573, .T. ) ;
#99991=ADVANCED_FACE ( 'NONE', ( #95391 ), #95997, .T. ) ;
#99992=CARTESIAN_POINT ( 'NONE',  ( 1.449999999999952216, 2.500000000000000000, -2.411473670974877859 ) ) ;
#99994=ORIENTED_EDGE ( 'NONE', *, *, #111115, .F. ) ;
#99995=DIRECTION ( 'NONE',  ( 0.000000000000000000, -0.9999939076577903929, 0.003490651415223739937 ) ) ;
#99996=DIRECTION ( 'NONE',  ( 0.000000000000000000, 0.000000000000000000, 1.000000000000000000 ) ) ;
#99997=DIRECTION ( 'NONE',  ( -0.000000000000000000, 1.000000000000000000, -0.000000000000000000 ) ) ;
#99998=DIRECTION ( 'NONE',  ( -0.000000000000000000, -1.000000000000000000, -0.000000000000000000 ) ) ;
#99999=VERTEX_POINT ( 'NONE', #43098 ) ;
#100000=CONICAL_SURFACE ( 'NONE', #102147, 0.1000000000000000472, 0.003490658503988666988 ) ;
#100001=DIRECTION ( 'NONE',  ( 0.000000000000000000, 0.000000000000000000, 1.000000000000000000 ) ) ;
#100002=CIRCLE ( 'NONE', #125132, 0.06509327318403745899 ) ;
#100003=ORIENTED_EDGE ( 'NONE', *, *, #43227, .T. ) ;
#100004=VERTEX_POINT ( 'NONE', #125489 ) ;
#100005=DIRECTION ( 'NONE',  ( 0.000000000000000000, 1.000000000000000000, 0.000000000000000000 ) ) ;
#100006=DIRECTION ( 'NONE',  ( 0.000000000000000000, 1.000000000000000000, 0.000000000000000000 ) ) ;
#100007=AXIS2_PLACEMENT_3D ( 'NONE', #93723, #121890, #61702 ) ;
#100008=ORIENTED_EDGE ( 'NONE', *, *, #58298, .F. ) ;
#100009=FACE_OUTER_BOUND ( 'NONE', #1648, .T. ) ;
#100010=FACE_OUTER_BOUND ( 'NONE', #128279, .T. ) ;
#100011=CARTESIAN_POINT ( 'NONE',  ( -2.500000000000030642, 12.50000000000000000, -0.6277270498435166823 ) ) ;
#100012=ORIENTED_EDGE ( 'NONE', *, *, #78276, .F. ) ;
#100013=CIRCLE ( 'NONE', #35186, 0.1000000000000002554 ) ;
#100014=PLANE ( 'NONE',  #82915 ) ;
#100015=ORIENTED_EDGE ( 'NONE', *, *, #5834, .F. ) ;
#100016=CARTESIAN_POINT ( 'NONE',  ( -1.900000000000034106, 12.50000000000000000, 0.4115034346978109769 ) ) ;
#100017=CIRCLE ( 'NONE', #70767, 0.09999999999999982514 ) ;
#100018=CONICAL_SURFACE ( 'NONE', #39405, 0.1000000000000000472, 0.003490658503988666988 ) ;
#100019=VERTEX_POINT ( 'NONE', #34561 ) ;
#100020=ADVANCED_FACE ( 'NONE', ( #14234 ), #14408, .T. ) ;
#100022=ORIENTED_EDGE ( 'NONE', *, *, #8198, .T. ) ;
#100023=DIRECTION ( 'NONE',  ( 0.000000000000000000, 0.000000000000000000, -1.000000000000000000 ) ) ;
#100024=CARTESIAN_POINT ( 'NONE',  ( -11.05000000000000249, 12.50000000000000000, -6.148780366869522673 ) ) ;
#100025=DIRECTION ( 'NONE',  ( 0.000000000000000000, 0.000000000000000000, 1.000000000000000000 ) ) ;
#100026=DIRECTION ( 'NONE',  ( -0.000000000000000000, -1.000000000000000000, -0.000000000000000000 ) ) ;
#100027=DIRECTION ( 'NONE',  ( 0.000000000000000000, 0.000000000000000000, 1.000000000000000000 ) ) ;
#100028=ORIENTED_EDGE ( 'NONE', *, *, #106869, .F. ) ;
#100029=ORIENTED_EDGE ( 'NONE', *, *, #90922, .T. ) ;
#100030=EDGE_CURVE ( 'NONE', #19145, #66592, #39593, .T. ) ;
#100031=ORIENTED_EDGE ( 'NONE', *, *, #123322, .F. ) ;
#100032=CARTESIAN_POINT ( 'NONE',  ( 15.59999999999988951, 2.500000000000000000, -0.3464101615137783474 ) ) ;
#100033=CARTESIAN_POINT ( 'NONE',  ( -12.09999999999999609, 12.50000000000000000, 0.6928203230275535862 ) ) ;
#100035=CONICAL_SURFACE ( 'NONE', #68628, 0.1000000000000000472, 0.003490658503988666988 ) ;
#100036=EDGE_LOOP ( 'NONE', ( #88476, #108995 ) ) ;
#100037=ORIENTED_EDGE ( 'NONE', *, *, #94826, .T. ) ;
#100038=ORIENTED_EDGE ( 'NONE', *, *, #11507, .F. ) ;
#100039=DIRECTION ( 'NONE',  ( 0.000000000000000000, 0.000000000000000000, 1.000000000000000000 ) ) ;
#100040=ORIENTED_EDGE ( 'NONE', *, *, #40074, .F. ) ;
#100042=VECTOR ( 'NONE', #49229, 1000.000000000000000 ) ;
#100043=DIRECTION ( 'NONE',  ( -0.000000000000000000, 1.000000000000000000, -0.000000000000000000 ) ) ;
#100044=CARTESIAN_POINT ( 'NONE',  ( 4.799999999999934097, 2.500000000000000000, 4.576537180435972019 ) ) ;
#100045=DIRECTION ( 'NONE',  ( -0.000000000000000000, -1.000000000000000000, -0.000000000000000000 ) ) ;
#100046=DIRECTION ( 'NONE',  ( 0.000000000000000000, -1.000000000000000000, 0.000000000000000000 ) ) ;
#100047=DIRECTION ( 'NONE',  ( -0.000000000000000000, -1.000000000000000000, -0.000000000000000000 ) ) ;
#100048=DIRECTION ( 'NONE',  ( 0.000000000000000000, 0.000000000000000000, 1.000000000000000000 ) ) ;
#100049=CIRCLE ( 'NONE', #112571, 0.1000000000000002554 ) ;
#100050=ORIENTED_EDGE ( 'NONE', *, *, #35991, .T. ) ;
#100051=AXIS2_PLACEMENT_3D ( 'NONE', #127717, #108074, #38061 ) ;
#100052=ORIENTED_EDGE ( 'NONE', *, *, #38032, .F. ) ;
#100053=CONICAL_SURFACE ( 'NONE', #125184, 0.09999999999999982514, 0.003490658503988666988 ) ;
#100054=DIRECTION ( 'NONE',  ( 0.000000000000000000, 0.000000000000000000, 1.000000000000000000 ) ) ;
#100055=AXIS2_PLACEMENT_3D ( 'NONE', #100334, #51251, #81341 ) ;
#100056=ORIENTED_EDGE ( 'NONE', *, *, #68777, .T. ) ;
#100057=VERTEX_POINT ( 'NONE', #103285 ) ;
#100059=CARTESIAN_POINT ( 'NONE',  ( 10.39999999999991331, 12.50000000000000000, -0.06509327318403980434 ) ) ;
#100060=CARTESIAN_POINT ( 'NONE',  ( -8.550000000000013145, 12.50000000000000000, -6.841600689897073373 ) ) ;
#100061=CIRCLE ( 'NONE', #47837, 0.09999999999999999167 ) ;
#100062=DIRECTION ( 'NONE',  ( 0.000000000000000000, 0.000000000000000000, 1.000000000000000000 ) ) ;
#100063=AXIS2_PLACEMENT_3D ( 'NONE', #77215, #8448, #69306 ) ;
#100064=EDGE_CURVE ( 'NONE', #114427, #82484, #74463, .T. ) ;
#100065=LINE ( 'NONE', #20855, #86695 ) ;
#100066=DIRECTION ( 'NONE',  ( 0.000000000000000000, 0.000000000000000000, 1.000000000000000000 ) ) ;
#100067=CARTESIAN_POINT ( 'NONE',  ( -2.500000000000031086, 2.500000000000000000, 3.737306695894644371 ) ) ;
#100068=CARTESIAN_POINT ( 'NONE',  ( 12.49999999999993960, 2.500000000000000000, 4.430127018922196847 ) ) ;
#100069=AXIS2_PLACEMENT_3D ( 'NONE', #6767, #101942, #75523 ) ;
#100070=EDGE_CURVE ( 'NONE', #5075, #38783, #1897, .T. ) ;
#100072=ORIENTED_EDGE ( 'NONE', *, *, #116237, .T. ) ;
#100073=CIRCLE ( 'NONE', #3922, 0.1000000000000000056 ) ;
#100076=ORIENTED_EDGE ( 'NONE', *, *, #31960, .F. ) ;
#100077=EDGE_CURVE ( 'NONE', #96401, #35080, #10314, .T. ) ;
#100078=CARTESIAN_POINT ( 'NONE',  ( 1.849999999999949685, 12.50000000000000000, -2.511473670974877948 ) ) ;
#100079=CARTESIAN_POINT ( 'NONE',  ( 0.8499999999999553468, 2.500000000000000000, 2.165063509461097713 ) ) ;
#100080=EDGE_LOOP ( 'NONE', ( #94016, #11641, #102403, #91873 ) ) ;
#100081=LINE ( 'NONE', #29413, #86233 ) ;
#100082=FACE_OUTER_BOUND ( 'NONE', #51568, .T. ) ;
#100084=ADVANCED_FACE ( 'NONE', ( #75108 ), #121034, .T. ) ;
#100085=DIRECTION ( 'NONE',  ( 0.000000000000000000, -0.000000000000000000, 1.000000000000000000 ) ) ;
#100086=DIRECTION ( 'NONE',  ( 0.000000000000000000, 1.000000000000000000, 0.000000000000000000 ) ) ;
#100087=ORIENTED_EDGE ( 'NONE', *, *, #71402, .F. ) ;
#100088=EDGE_CURVE ( 'NONE', #6835, #38646, #85526, .T. ) ;
#100089=DIRECTION ( 'NONE',  ( -0.000000000000000000, 1.000000000000000000, -0.000000000000000000 ) ) ;
#100090=AXIS2_PLACEMENT_3D ( 'NONE', #211, #19881, #8739 ) ;
#100091=VECTOR ( 'NONE', #53329, 1000.000000000000000 ) ;
#100092=DIRECTION ( 'NONE',  ( 0.000000000000000000, 1.000000000000000000, 0.000000000000000000 ) ) ;
#100093=ORIENTED_EDGE ( 'NONE', *, *, #70663, .F. ) ;
#100094=CIRCLE ( 'NONE', #31153, 0.1000000000000002554 ) ;
#100095=EDGE_LOOP ( 'NONE', ( #36413, #98390, #127348, #77144 ) ) ;
#100096=EDGE_LOOP ( 'NONE', ( #123232, #19054 ) ) ;
#100097=ORIENTED_EDGE ( 'NONE', *, *, #41922, .T. ) ;
#100098=CARTESIAN_POINT ( 'NONE',  ( 0.1999999999999627909, 2.500000000000000000, 0.2464101615137758439 ) ) ;
#100099=AXIS2_PLACEMENT_3D ( 'NONE', #24520, #93909, #46096 ) ;
#100101=DIRECTION ( 'NONE',  ( -0.000000000000000000, -1.000000000000000000, -0.000000000000000000 ) ) ;
#100102=CIRCLE ( 'NONE', #54401, 0.1000000000000002554 ) ;
#100104=CARTESIAN_POINT ( 'NONE',  ( -2.900000000000030109, 2.500000000000000000, 0.5928203230275495006 ) ) ;
#100105=EDGE_LOOP ( 'NONE', ( #100660, #83313 ) ) ;
#100106=DIRECTION ( 'NONE',  ( -0.000000000000000000, 1.000000000000000000, -0.000000000000000000 ) ) ;
#100107=CARTESIAN_POINT ( 'NONE',  ( -9.600000000000008527, 12.50000000000000000, -2.385244779468109755E-15 ) ) ;
#100108=AXIS2_PLACEMENT_3D ( 'NONE', #470, #91446, #80352 ) ;
#100109=DIRECTION ( 'NONE',  ( 0.000000000000000000, 0.000000000000000000, 1.000000000000000000 ) ) ;
#100110=CARTESIAN_POINT ( 'NONE',  ( -7.300000000000013145, 2.500000000000000000, 3.983716857408420076 ) ) ;
#100111=ORIENTED_EDGE ( 'NONE', *, *, #108820, .F. ) ;
#100112=AXIS2_PLACEMENT_3D ( 'NONE', #61439, #119682, #100682 ) ;
#100113=CONICAL_SURFACE ( 'NONE', #16464, 0.09999999999999982514, 0.003490658503988666988 ) ;
#100115=ORIENTED_EDGE ( 'NONE', *, *, #116236, .F. ) ;
#100116=EDGE_LOOP ( 'NONE', ( #54096, #6937, #77625, #4526 ) ) ;
#100117=PLANE ( 'NONE',  #74833 ) ;
#100118=LINE ( 'NONE', #11066, #18852 ) ;
#100119=FACE_BOUND ( 'NONE', #5549, .T. ) ;
#100120=CARTESIAN_POINT ( 'NONE',  ( -6.250000000000019540, 2.500000000000000000, -7.188010851410854052 ) ) ;
#100121=CARTESIAN_POINT ( 'NONE',  ( 11.24999999999990585, 12.50000000000000000, -5.802370205355749988 ) ) ;
#100122=CARTESIAN_POINT ( 'NONE',  ( 5.649999999999934630, 12.50000000000000000, 6.906693963081109722 ) ) ;
#100123=EDGE_CURVE ( 'NONE', #55074, #64406, #81335, .T. ) ;
#100124=CONICAL_SURFACE ( 'NONE', #116828, 0.1000000000000002554, 0.003490658503988666988 ) ;
#100125=EDGE_CURVE ( 'NONE', #93392, #110307, #112728, .T. ) ;
#100126=CARTESIAN_POINT ( 'NONE',  ( 9.599999999999917932, 2.500000000000000000, 0.09999999999999772959 ) ) ;
#100127=DIRECTION ( 'NONE',  ( 0.000000000000000000, 0.000000000000000000, 1.000000000000000000 ) ) ;
#100128=CARTESIAN_POINT ( 'NONE',  ( -0.4000000000000392131, 12.50000000000000000, -4.330127018922201643 ) ) ;
#100129=ADVANCED_FACE ( 'NONE', ( #56097 ), #129475, .T. ) ;
#100131=ORIENTED_EDGE ( 'NONE', *, *, #113142, .T. ) ;
#100132=ADVANCED_FACE ( 'NONE', ( #36492 ), #93844, .T. ) ;
#100133=DIRECTION ( 'NONE',  ( 0.000000000000000000, 0.000000000000000000, 1.000000000000000000 ) ) ;
#100134=CIRCLE ( 'NONE', #18557, 0.06509327318403745899 ) ;
#100135=AXIS2_PLACEMENT_3D ( 'NONE', #52903, #39875, #100695 ) ;
#100136=CARTESIAN_POINT ( 'NONE',  ( 9.999999999999912959, 2.500000000000000000, -5.122947341949753763 ) ) ;
#100137=EDGE_CURVE ( 'NONE', #4249, #93494, #27040, .T. ) ;
#100138=ORIENTED_EDGE ( 'NONE', *, *, #118111, .T. ) ;
#100139=VERTEX_POINT ( 'NONE', #7638 ) ;
#100142=FACE_BOUND ( 'NONE', #111810, .T. ) ;
#100143=CARTESIAN_POINT ( 'NONE',  ( 10.61495711629423155, -2.500000000000001332, -8.020491763388223561 ) ) ;
#100144=AXIS2_PLACEMENT_3D ( 'NONE', #107641, #106972, #67042 ) ;
#100145=CIRCLE ( 'NONE', #35306, 0.06509327318403745899 ) ;
#100146=EDGE_CURVE ( 'NONE', #60649, #15598, #77042, .T. ) ;
#100147=AXIS2_PLACEMENT_3D ( 'NONE', #19366, #88094, #78327 ) ;
#100148=ADVANCED_FACE ( 'NONE', ( #86188 ), #60602, .T. ) ;
#100149=DIRECTION ( 'NONE',  ( -0.000000000000000000, -1.000000000000000000, -0.000000000000000000 ) ) ;
#100150=ORIENTED_EDGE ( 'NONE', *, *, #43814, .F. ) ;
#100151=DIRECTION ( 'NONE',  ( 0.000000000000000000, 0.000000000000000000, 1.000000000000000000 ) ) ;
#100152=CARTESIAN_POINT ( 'NONE',  ( -4.076600168545496672E-14, 2.500000000000000000, -5.022947341949754119 ) ) ;
#100153=CIRCLE ( 'NONE', #60464, 0.06509327318403745899 ) ;
#100154=ORIENTED_EDGE ( 'NONE', *, *, #21341, .F. ) ;
#100156=DIRECTION ( 'NONE',  ( 0.000000000000000000, 0.000000000000000000, 1.000000000000000000 ) ) ;
#100157=AXIS2_PLACEMENT_3D ( 'NONE', #51630, #111834, #62098 ) ;
#100158=CARTESIAN_POINT ( 'NONE',  ( 0.8499999999999553468, 12.50000000000000000, 2.165063509461097713 ) ) ;
#100159=FACE_OUTER_BOUND ( 'NONE', #25293, .T. ) ;
#100160=ORIENTED_EDGE ( 'NONE', *, *, #6502, .T. ) ;
#100161=LINE ( 'NONE', #41254, #121935 ) ;
#100162=CARTESIAN_POINT ( 'NONE',  ( -3.749999999999991562, 2.500000000000000000, 6.495190528383297135 ) ) ;
#100163=DIRECTION ( 'NONE',  ( 0.000000000000000000, -0.000000000000000000, 1.000000000000000000 ) ) ;
#100164=AXIS2_PLACEMENT_3D ( 'NONE', #65720, #116745, #95833 ) ;
#100165=DIRECTION ( 'NONE',  ( 0.000000000000000000, 0.000000000000000000, 1.000000000000000000 ) ) ;
#100166=ORIENTED_EDGE ( 'NONE', *, *, #111453, .F. ) ;
#100167=ORIENTED_EDGE ( 'NONE', *, *, #62722, .T. ) ;
#100168=ADVANCED_FACE ( 'NONE', ( #108423 ), #24981, .T. ) ;
#100169=DIRECTION ( 'NONE',  ( 0.000000000000000000, -0.000000000000000000, 1.000000000000000000 ) ) ;
#100170=VERTEX_POINT ( 'NONE', #128746 ) ;
#100171=DIRECTION ( 'NONE',  ( 0.000000000000000000, -0.9999939076577903929, 0.003490651415223739937 ) ) ;
#100172=DIRECTION ( 'NONE',  ( -4.274815082592931898E-19, -0.9999939076577903929, -0.003490651415223739937 ) ) ;
#100173=CARTESIAN_POINT ( 'NONE',  ( -14.59999999999998366, 2.500000000000000000, 0.5928203230275517210 ) ) ;
#100174=VERTEX_POINT ( 'NONE', #18107 ) ;
#100175=DIRECTION ( 'NONE',  ( -4.274815082592931898E-19, -0.9999939076577903929, -0.003490651415223739937 ) ) ;
#100176=CARTESIAN_POINT ( 'NONE',  ( -15.79999999999998117, 12.50000000000000000, 0.000000000000000000 ) ) ;
#100177=DIRECTION ( 'NONE',  ( -0.000000000000000000, -1.000000000000000000, -0.000000000000000000 ) ) ;
#100178=DIRECTION ( 'NONE',  ( 0.000000000000000000, 1.000000000000000000, 0.000000000000000000 ) ) ;
#100179=LINE ( 'NONE', #28217, #31943 ) ;
#100180=CIRCLE ( 'NONE', #31237, 0.1000000000000002554 ) ;
#100181=FACE_OUTER_BOUND ( 'NONE', #10915, .T. ) ;
#100182=CIRCLE ( 'NONE', #33299, 0.06509327318403745899 ) ;
#100183=VERTEX_POINT ( 'NONE', #58054 ) ;
#100185=ORIENTED_EDGE ( 'NONE', *, *, #42610, .F. ) ;
#100186=DIRECTION ( 'NONE',  ( 0.000000000000000000, 0.000000000000000000, 1.000000000000000000 ) ) ;
#100187=ORIENTED_EDGE ( 'NONE', *, *, #95830, .T. ) ;
#100188=DIRECTION ( 'NONE',  ( -0.000000000000000000, 1.000000000000000000, -0.000000000000000000 ) ) ;
#100189=EDGE_LOOP ( 'NONE', ( #35908, #72389, #34002, #123990 ) ) ;
#100190=ORIENTED_EDGE ( 'NONE', *, *, #72215, .F. ) ;
#100191=ORIENTED_EDGE ( 'NONE', *, *, #67560, .T. ) ;
#100192=CONICAL_SURFACE ( 'NONE', #60497, 0.1000000000000002554, 0.003490658503988666988 ) ;
#100193=LINE ( 'NONE', #30175, #20723 ) ;
#100194=CARTESIAN_POINT ( 'NONE',  ( -4.400000000000028777, 2.500000000000000000, -4.576537180435978236 ) ) ;
#100195=DIRECTION ( 'NONE',  ( 0.000000000000000000, 0.000000000000000000, -1.000000000000000000 ) ) ;
#100197=VECTOR ( 'NONE', #119543, 1000.000000000000000 ) ;
#100198=CARTESIAN_POINT ( 'NONE',  ( -0.6000000000000323963, 12.50000000000000000, -0.4115034346978133639 ) ) ;
#100199=LINE ( 'NONE', #49823, #121144 ) ;
#100200=DIRECTION ( 'NONE',  ( -0.000000000000000000, 1.000000000000000000, -0.000000000000000000 ) ) ;
#100201=CARTESIAN_POINT ( 'NONE',  ( 12.29999999999990479, 2.500000000000000000, -4.083716857408426826 ) ) ;
#100202=CARTESIAN_POINT ( 'NONE',  ( 6.649999999999931966, 2.500000000000000000, -7.188010851410854052 ) ) ;
#100203=VECTOR ( 'NONE', #24492, 1000.000000000000000 ) ;
#100204=DIRECTION ( 'NONE',  ( 0.000000000000000000, 0.000000000000000000, 1.000000000000000000 ) ) ;
#100205=AXIS2_PLACEMENT_3D ( 'NONE', #88112, #37759, #128077 ) ;
#100206=AXIS2_PLACEMENT_3D ( 'NONE', #56134, #69169, #10273 ) ;
#100207=EDGE_LOOP ( 'NONE', ( #45178, #67750 ) ) ;
#100208=DIRECTION ( 'NONE',  ( 0.000000000000000000, 1.000000000000000000, 0.000000000000000000 ) ) ;
#100209=ORIENTED_EDGE ( 'NONE', *, *, #109392, .T. ) ;
#100210=ORIENTED_EDGE ( 'NONE', *, *, #83457, .T. ) ;
#100211=CARTESIAN_POINT ( 'NONE',  ( 8.749999999999953815, 2.500000000000000000, -2.265063509461101798 ) ) ;
#100212=DIRECTION ( 'NONE',  ( 0.000000000000000000, 0.000000000000000000, 1.000000000000000000 ) ) ;
#100213=CARTESIAN_POINT ( 'NONE',  ( 8.099999999999923261, 12.50000000000000000, -4.676537180435978769 ) ) ;
#100214=FACE_OUTER_BOUND ( 'NONE', #107983, .T. ) ;
#100215=CARTESIAN_POINT ( 'NONE',  ( 1.049999999999954081, 2.500000000000000000, -6.248780366869526759 ) ) ;
#100216=DIRECTION ( 'NONE',  ( 0.000000000000000000, -0.9999939076577903929, 0.003490651415223739937 ) ) ;
#100217=AXIS2_PLACEMENT_3D ( 'NONE', #88877, #12085, #61196 ) ;
#100218=ORIENTED_EDGE ( 'NONE', *, *, #82968, .F. ) ;
#100219=ORIENTED_EDGE ( 'NONE', *, *, #111436, .F. ) ;
#100220=AXIS2_PLACEMENT_3D ( 'NONE', #120698, #70956, #21204 ) ;
#100221=DIRECTION ( 'NONE',  ( 0.000000000000000000, 0.000000000000000000, -1.000000000000000000 ) ) ;
#100222=EDGE_CURVE ( 'NONE', #62914, #53677, #79370, .T. ) ;
#100223=AXIS2_PLACEMENT_3D ( 'NONE', #93473, #3796, #103936 ) ;
#100224=ORIENTED_EDGE ( 'NONE', *, *, #92005, .F. ) ;
#100225=FACE_OUTER_BOUND ( 'NONE', #74340, .T. ) ;
#100226=ORIENTED_EDGE ( 'NONE', *, *, #93211, .T. ) ;
#100227=EDGE_CURVE ( 'NONE', #67249, #86863, #66559, .T. ) ;
#100228=ORIENTED_EDGE ( 'NONE', *, *, #73044, .F. ) ;
#100229=EDGE_CURVE ( 'NONE', #122300, #28419, #16644, .T. ) ;
#100230=PLANE ( 'NONE',  #69089 ) ;
#100231=AXIS2_PLACEMENT_3D ( 'NONE', #57083, #125816, #5406 ) ;
#100232=DIRECTION ( 'NONE',  ( -0.000000000000000000, 1.000000000000000000, -0.000000000000000000 ) ) ;
#100233=AXIS2_PLACEMENT_3D ( 'NONE', #36481, #56712, #107773 ) ;
#100234=AXIS2_PLACEMENT_3D ( 'NONE', #36119, #36773, #5988 ) ;
#100235=DIRECTION ( 'NONE',  ( -0.000000000000000000, 1.000000000000000000, -0.000000000000000000 ) ) ;
#100236=CARTESIAN_POINT ( 'NONE',  ( -4.150000000000024336, 2.500000000000000000, -2.265063509461101798 ) ) ;
#100237=EDGE_CURVE ( 'NONE', #6356, #2890, #28588, .T. ) ;
#100238=FACE_OUTER_BOUND ( 'NONE', #84718, .T. ) ;
#100239=EDGE_CURVE ( 'NONE', #11222, #108234, #6978, .T. ) ;
#100240=ORIENTED_EDGE ( 'NONE', *, *, #109734, .F. ) ;
#100241=DIRECTION ( 'NONE',  ( 0.000000000000000000, -0.000000000000000000, 1.000000000000000000 ) ) ;
#100242=CARTESIAN_POINT ( 'NONE',  ( -3.100000000000028511, 2.500000000000000000, -0.3464101615137782364 ) ) ;
#100243=EDGE_CURVE ( 'NONE', #127840, #110110, #64685, .T. ) ;
#100244=DIRECTION ( 'NONE',  ( 0.000000000000000000, 1.000000000000000000, 0.000000000000000000 ) ) ;
#100245=EDGE_CURVE ( 'NONE', #18590, #75910, #37125, .T. ) ;
#100246=ADVANCED_FACE ( 'NONE', ( #67180 ), #116990, .T. ) ;
#100247=DIRECTION ( 'NONE',  ( 0.000000000000000000, -0.000000000000000000, 1.000000000000000000 ) ) ;
#100248=CIRCLE ( 'NONE', #102389, 0.09999999999999982514 ) ;
#100249=DIRECTION ( 'NONE',  ( 0.000000000000000000, 0.000000000000000000, 1.000000000000000000 ) ) ;
#100250=CIRCLE ( 'NONE', #35403, 0.1000000000000002554 ) ;
#100251=ORIENTED_EDGE ( 'NONE', *, *, #78978, .F. ) ;
#100252=CIRCLE ( 'NONE', #35505, 0.06509327318403745899 ) ;
#100253=ORIENTED_EDGE ( 'NONE', *, *, #14401, .F. ) ;
#100254=FACE_OUTER_BOUND ( 'NONE', #121469, .T. ) ;
#100255=ADVANCED_FACE ( 'NONE', ( #107125 ), #47979, .T. ) ;
#100256=ORIENTED_EDGE ( 'NONE', *, *, #124639, .T. ) ;
#100257=CARTESIAN_POINT ( 'NONE',  ( 17.50000000000000355, -2.413248583741843589, 3.595440551767155934 ) ) ;
#100258=DIRECTION ( 'NONE',  ( 0.000000000000000000, 0.000000000000000000, 1.000000000000000000 ) ) ;
#100259=CIRCLE ( 'NONE', #83538, 0.06509327318403745899 ) ;
#100261=CARTESIAN_POINT ( 'NONE',  ( 2.499999999999947153, 12.50000000000000000, 3.637306695894644726 ) ) ;
#100262=DIRECTION ( 'NONE',  ( 0.000000000000000000, 0.000000000000000000, 1.000000000000000000 ) ) ;
#100263=DIRECTION ( 'NONE',  ( 0.000000000000000000, 0.000000000000000000, -1.000000000000000000 ) ) ;
#100264=DIRECTION ( 'NONE',  ( 0.000000000000000000, -0.9999939076577903929, 0.003490651415223739937 ) ) ;
#100265=DIRECTION ( 'NONE',  ( 0.000000000000000000, 0.000000000000000000, -1.000000000000000000 ) ) ;
#100266=VERTEX_POINT ( 'NONE', #8922 ) ;
#100268=CARTESIAN_POINT ( 'NONE',  ( 21.24754738303275658, 0.7337760880902297611, -4.182111650399359171 ) ) ;
#100269=DIRECTION ( 'NONE',  ( -4.274815082592931898E-19, -0.9999939076577903929, -0.003490651415223739937 ) ) ;
#100270=DIRECTION ( 'NONE',  ( 0.000000000000000000, 0.000000000000000000, 1.000000000000000000 ) ) ;
#100271=DIRECTION ( 'NONE',  ( -0.000000000000000000, 1.000000000000000000, -0.000000000000000000 ) ) ;
#100272=ORIENTED_EDGE ( 'NONE', *, *, #9492, .F. ) ;
#100273=ORIENTED_EDGE ( 'NONE', *, *, #122437, .T. ) ;
#100274=EDGE_CURVE ( 'NONE', #43147, #108043, #129567, .T. ) ;
#100275=CARTESIAN_POINT ( 'NONE',  ( -1.450000000000035039, 2.500000000000000000, -2.511473670974877948 ) ) ;
#100276=CIRCLE ( 'NONE', #8319, 0.1000000000000000472 ) ;
#100277=DIRECTION ( 'NONE',  ( 0.000000000000000000, 0.000000000000000000, 1.000000000000000000 ) ) ;
#100278=DIRECTION ( 'NONE',  ( 0.000000000000000000, 0.000000000000000000, 1.000000000000000000 ) ) ;
#100279=EDGE_CURVE ( 'NONE', #93088, #119152, #6185, .T. ) ;
#100280=ORIENTED_EDGE ( 'NONE', *, *, #70743, .F. ) ;
#100281=DIRECTION ( 'NONE',  ( 0.000000000000000000, 1.000000000000000000, 0.000000000000000000 ) ) ;
#100282=EDGE_CURVE ( 'NONE', #40877, #76430, #12450, .T. ) ;
#100283=VECTOR ( 'NONE', #54664, 1000.000000000000000 ) ;
#100284=CONICAL_SURFACE ( 'NONE', #102436, 0.09999999999999982514, 0.003490658503988666988 ) ;
#100285=DIRECTION ( 'NONE',  ( -4.274815082592931898E-19, -0.9999939076577903929, -0.003490651415223739937 ) ) ;
#100286=CIRCLE ( 'NONE', #112810, 0.06509327318403745899 ) ;
#100287=ORIENTED_EDGE ( 'NONE', *, *, #16331, .F. ) ;
#100288=CARTESIAN_POINT ( 'NONE',  ( 10.64999999999990976, 2.500000000000000000, -6.941600689897077459 ) ) ;
#100290=ORIENTED_EDGE ( 'NONE', *, *, #97607, .T. ) ;
#100292=ADVANCED_FACE ( 'NONE', ( #89435 ), #75161, .T. ) ;
#100293=AXIS2_PLACEMENT_3D ( 'NONE', #97960, #118248, #58690 ) ;
#100294=AXIS2_PLACEMENT_3D ( 'NONE', #25225, #66450, #57939 ) ;
#100295=ADVANCED_FACE ( 'NONE', ( #90064 ), #93944, .T. ) ;
#100296=EDGE_CURVE ( 'NONE', #73598, #109355, #49525, .T. ) ;
#100297=ORIENTED_EDGE ( 'NONE', *, *, #110866, .T. ) ;
#100298=DIRECTION ( 'NONE',  ( 0.000000000000000000, 0.000000000000000000, 1.000000000000000000 ) ) ;
#100299=CARTESIAN_POINT ( 'NONE',  ( 15.62915144542244583, 2.499999999999999556, -5.624002559040090610 ) ) ;
#100300=ORIENTED_EDGE ( 'NONE', *, *, #36832, .F. ) ;
#100301=ORIENTED_EDGE ( 'NONE', *, *, #45253, .F. ) ;
#100302=DIRECTION ( 'NONE',  ( 0.000000000000000000, 1.000000000000000000, 0.000000000000000000 ) ) ;
#100303=CARTESIAN_POINT ( 'NONE',  ( 11.89999999999990798, 2.500000000000000000, -4.676537180435977881 ) ) ;
#100304=ORIENTED_EDGE ( 'NONE', *, *, #117221, .T. ) ;
#100305=EDGE_CURVE ( 'NONE', #13873, #91647, #123278, .T. ) ;
#100306=CARTESIAN_POINT ( 'NONE',  ( -5.000000000000022204, 12.50000000000000000, -0.6928203230275541413 ) ) ;
#100308=CARTESIAN_POINT ( 'NONE',  ( 4.599999999999936584, 2.500000000000000000, 3.637306695894644726 ) ) ;
#100310=CARTESIAN_POINT ( 'NONE',  ( -5.400000000000020783, 12.50000000000000000, 5.022947341949748790 ) ) ;
#100311=CARTESIAN_POINT ( 'NONE',  ( 4.999999999999973355, 12.50000000000000000, -4.330127018922201643 ) ) ;
#100312=PLANE ( 'NONE',  #100603 ) ;
#100313=VECTOR ( 'NONE', #21870, 1000.000000000000000 ) ;
#100314=CIRCLE ( 'NONE', #27059, 0.09999999999999982514 ) ;
#100315=ORIENTED_EDGE ( 'NONE', *, *, #56331, .T. ) ;
#100316=EDGE_LOOP ( 'NONE', ( #67658, #40834, #102273, #53682 ) ) ;
#100317=ORIENTED_EDGE ( 'NONE', *, *, #75095, .T. ) ;
#100318=CARTESIAN_POINT ( 'NONE',  ( -10.84999999999999964, 12.50000000000000000, 7.188010851410848723 ) ) ;
#100319=PLANE ( 'NONE',  #57493 ) ;
#100320=CARTESIAN_POINT ( 'NONE',  ( 10.84999999999991260, 2.500000000000000000, 5.802370205355744659 ) ) ;
#100321=EDGE_LOOP ( 'NONE', ( #46995, #88553 ) ) ;
#100322=ORIENTED_EDGE ( 'NONE', *, *, #15389, .T. ) ;
#100323=FACE_BOUND ( 'NONE', #118699, .T. ) ;
#100324=VERTEX_POINT ( 'NONE', #21333 ) ;
#100325=EDGE_CURVE ( 'NONE', #6598, #67150, #110360, .T. ) ;
#100326=DIRECTION ( 'NONE',  ( 0.000000000000000000, 0.000000000000000000, 1.000000000000000000 ) ) ;
#100327=CARTESIAN_POINT ( 'NONE',  ( -4.293440603042597559E-14, 2.500000000000000000, 5.022947341949748790 ) ) ;
#100328=CIRCLE ( 'NONE', #31290, 0.09999999999999982514 ) ;
#100329=CARTESIAN_POINT ( 'NONE',  ( -5.400000000000020783, 12.50000000000000000, 5.088040615133786027 ) ) ;
#100330=CARTESIAN_POINT ( 'NONE',  ( -1.250000000000036193, 12.50000000000000000, 1.472243186433545459 ) ) ;
#100331=CARTESIAN_POINT ( 'NONE',  ( -11.25000000000000000, 2.500000000000000000, -7.088010851410849966 ) ) ;
#100332=DIRECTION ( 'NONE',  ( -0.000000000000000000, 1.000000000000000000, -0.000000000000000000 ) ) ;
#100333=CARTESIAN_POINT ( 'NONE',  ( 13.94999999999989804, 12.50000000000000000, 1.753560074763284016 ) ) ;
#100334=CARTESIAN_POINT ( 'NONE',  ( 11.64999999999990443, 2.500000000000000000, 1.472243186433545459 ) ) ;
#100335=LINE ( 'NONE', #33536, #57959 ) ;
#100336=CIRCLE ( 'NONE', #31390, 0.09999999999999982514 ) ;
#100337=DIRECTION ( 'NONE',  ( 0.000000000000000000, 0.000000000000000000, 1.000000000000000000 ) ) ;
#100338=ORIENTED_EDGE ( 'NONE', *, *, #24868, .F. ) ;
#100339=EDGE_LOOP ( 'NONE', ( #36460, #84797, #77715, #40125 ) ) ;
#100340=CIRCLE ( 'NONE', #43914, 0.09999999999999982514 ) ;
#100341=EDGE_CURVE ( 'NONE', #118072, #107774, #112817, .T. ) ;
#100342=ORIENTED_EDGE ( 'NONE', *, *, #17438, .F. ) ;
#100343=ORIENTED_EDGE ( 'NONE', *, *, #39698, .T. ) ;
#100345=CARTESIAN_POINT ( 'NONE',  ( -8.550000000000013145, 2.500000000000000000, -1.718653347947326049 ) ) ;
#100346=DIRECTION ( 'NONE',  ( 0.000000000000000000, 1.000000000000000000, 0.000000000000000000 ) ) ;
#100347=EDGE_LOOP ( 'NONE', ( #99803, #5542 ) ) ;
#100348=VERTEX_POINT ( 'NONE', #91367 ) ;
#100349=AXIS2_PLACEMENT_3D ( 'NONE', #77948, #118514, #87122 ) ;
#100350=ORIENTED_EDGE ( 'NONE', *, *, #14133, .F. ) ;
#100351=LINE ( 'NONE', #1486, #27101 ) ;
#100352=VECTOR ( 'NONE', #15545, 1000.000000000000000 ) ;
#100353=DIRECTION ( 'NONE',  ( 0.000000000000000000, 1.000000000000000000, 0.000000000000000000 ) ) ;
#100355=DIRECTION ( 'NONE',  ( 0.000000000000000000, 1.000000000000000000, 0.000000000000000000 ) ) ;
#100356=DIRECTION ( 'NONE',  ( 0.000000000000000000, 1.000000000000000000, 0.000000000000000000 ) ) ;
#100357=AXIS2_PLACEMENT_3D ( 'NONE', #19646, #59595, #20930 ) ;
#100358=DIRECTION ( 'NONE',  ( 0.000000000000000000, 0.000000000000000000, -1.000000000000000000 ) ) ;
#100359=DIRECTION ( 'NONE',  ( 0.000000000000000000, 0.000000000000000000, -1.000000000000000000 ) ) ;
#100361=EDGE_LOOP ( 'NONE', ( #821, #87587 ) ) ;
#100362=DIRECTION ( 'NONE',  ( 0.000000000000000000, 0.000000000000000000, 1.000000000000000000 ) ) ;
#100363=VERTEX_POINT ( 'NONE', #50645 ) ;
#100364=ORIENTED_EDGE ( 'NONE', *, *, #116746, .F. ) ;
#100367=EDGE_LOOP ( 'NONE', ( #53713, #127356, #114370, #100219 ) ) ;
#100368=EDGE_LOOP ( 'NONE', ( #106361, #22422 ) ) ;
#100369=CARTESIAN_POINT ( 'NONE',  ( 9.149999999999918643, 2.500000000000000000, -6.595190528383302109 ) ) ;
#100370=DIRECTION ( 'NONE',  ( -0.000000000000000000, -1.000000000000000000, -0.000000000000000000 ) ) ;
#100371=CARTESIAN_POINT ( 'NONE',  ( -2.100000000000034284, 2.500000000000000000, -4.330127018922201643 ) ) ;
#100372=CARTESIAN_POINT ( 'NONE',  ( 13.09999999999990195, 2.500000000000000000, 3.983716857408420076 ) ) ;
#100373=CARTESIAN_POINT ( 'NONE',  ( -12.09999999999999609, 2.500000000000000000, -5.022947341949751454 ) ) ;
#100374=LINE ( 'NONE', #50619, #77594 ) ;
#100375=LINE ( 'NONE', #90544, #51321 ) ;
#100376=ORIENTED_EDGE ( 'NONE', *, *, #91979, .F. ) ;
#100377=LINE ( 'NONE', #48708, #115217 ) ;
#100378=EDGE_CURVE ( 'NONE', #50211, #54998, #120039, .T. ) ;
#100379=VECTOR ( 'NONE', #31090, 1000.000000000000000 ) ;
#100380=EDGE_LOOP ( 'NONE', ( #5083, #123326, #19001, #31622 ) ) ;
#100381=CARTESIAN_POINT ( 'NONE',  ( -6.250000000000017764, 2.500000000000000000, 7.188010851410848723 ) ) ;
#100382=CARTESIAN_POINT ( 'NONE',  ( -7.500000000000001776, 1.500000000000000000, 10.00000000000000178 ) ) ;
#100383=ORIENTED_EDGE ( 'NONE', *, *, #51119, .F. ) ;
#100384=FACE_OUTER_BOUND ( 'NONE', #106808, .T. ) ;
#100385=DIRECTION ( 'NONE',  ( -0.000000000000000000, 1.000000000000000000, -0.000000000000000000 ) ) ;
#100386=ORIENTED_EDGE ( 'NONE', *, *, #110150, .F. ) ;
#100387=EDGE_CURVE ( 'NONE', #35157, #62991, #101686, .T. ) ;
#100388=AXIS2_PLACEMENT_3D ( 'NONE', #57748, #38099, #55801 ) ;
#100389=LINE ( 'NONE', #32321, #15398 ) ;
#100390=ORIENTED_EDGE ( 'NONE', *, *, #4896, .F. ) ;
#100391=EDGE_CURVE ( 'NONE', #38596, #89563, #33412, .T. ) ;
#100392=EDGE_CURVE ( 'NONE', #88710, #61895, #243, .T. ) ;
#100393=ORIENTED_EDGE ( 'NONE', *, *, #77407, .F. ) ;
#100394=LINE ( 'NONE', #60488, #14281 ) ;
#100395=DIRECTION ( 'NONE',  ( 0.000000000000000000, 0.000000000000000000, -1.000000000000000000 ) ) ;
#100396=ADVANCED_FACE ( 'NONE', ( #69641 ), #83580, .T. ) ;
#100397=DIRECTION ( 'NONE',  ( -4.274815082592931898E-19, -0.9999939076577903929, -0.003490651415223739937 ) ) ;
#100398=ADVANCED_FACE ( 'NONE', ( #19234 ), #59195, .T. ) ;
#100399=DIRECTION ( 'NONE',  ( 0.000000000000000000, 1.000000000000000000, 0.000000000000000000 ) ) ;
#100400=DIRECTION ( 'NONE',  ( 0.000000000000000000, -0.000000000000000000, 1.000000000000000000 ) ) ;
#100401=VERTEX_POINT ( 'NONE', #99759 ) ;
#100402=DIRECTION ( 'NONE',  ( -0.000000000000000000, -1.000000000000000000, -0.000000000000000000 ) ) ;
#100403=EDGE_CURVE ( 'NONE', #62801, #115200, #20549, .T. ) ;
#100404=VERTEX_POINT ( 'NONE', #10692 ) ;
#100405=EDGE_CURVE ( 'NONE', #26161, #63939, #90564, .T. ) ;
#100406=DIRECTION ( 'NONE',  ( 0.000000000000000000, 0.000000000000000000, 1.000000000000000000 ) ) ;
#100407=CIRCLE ( 'NONE', #58556, 0.1000000000000000472 ) ;
#100408=DIRECTION ( 'NONE',  ( 0.000000000000000000, 0.000000000000000000, 1.000000000000000000 ) ) ;
#100409=EDGE_CURVE ( 'NONE', #58364, #2839, #21181, .T. ) ;
#100410=VECTOR ( 'NONE', #84053, 1000.000000000000000 ) ;
#100412=DIRECTION ( 'NONE',  ( 0.000000000000000000, -0.000000000000000000, 1.000000000000000000 ) ) ;
#100413=CARTESIAN_POINT ( 'NONE',  ( 2.299999999999948752, 2.500000000000000000, -3.883716857408426648 ) ) ;
#100414=CARTESIAN_POINT ( 'NONE',  ( 8.149999999999920419, 12.50000000000000000, -1.753560074763288457 ) ) ;
#100415=DIRECTION ( 'NONE',  ( 0.000000000000000000, -0.000000000000000000, 1.000000000000000000 ) ) ;
#100416=ORIENTED_EDGE ( 'NONE', *, *, #23218, .T. ) ;
#100417=VECTOR ( 'NONE', #10423, 1000.000000000000000 ) ;
#100418=FACE_OUTER_BOUND ( 'NONE', #26956, .T. ) ;
#100419=DIRECTION ( 'NONE',  ( -0.000000000000000000, -1.000000000000000000, -0.000000000000000000 ) ) ;
#100420=DIRECTION ( 'NONE',  ( 0.000000000000000000, 0.000000000000000000, -1.000000000000000000 ) ) ;
#100421=ORIENTED_EDGE ( 'NONE', *, *, #39860, .T. ) ;
#100422=CARTESIAN_POINT ( 'NONE',  ( 2.499999999999947153, 2.500000000000000000, 0.6928203230275494784 ) ) ;
#100423=CONICAL_SURFACE ( 'NONE', #115069, 0.1000000000000002554, 0.003490658503988666988 ) ;
#100424=AXIS2_PLACEMENT_3D ( 'NONE', #29294, #98649, #9641 ) ;
#100425=EDGE_LOOP ( 'NONE', ( #57139, #7633 ) ) ;
#100426=VERTEX_POINT ( 'NONE', #103623 ) ;
#100427=DIRECTION ( 'NONE',  ( -0.000000000000000000, -1.000000000000000000, -0.000000000000000000 ) ) ;
#100428=ORIENTED_EDGE ( 'NONE', *, *, #61887, .T. ) ;
#100429=DIRECTION ( 'NONE',  ( -4.274815082592931898E-19, -0.9999939076577903929, -0.003490651415223739937 ) ) ;
#100430=CARTESIAN_POINT ( 'NONE',  ( 3.349999999999941913, 12.50000000000000000, 5.867463478539781896 ) ) ;
#100431=VECTOR ( 'NONE', #128297, 1000.000000000000000 ) ;
#100433=DIRECTION ( 'NONE',  ( 0.000000000000000000, 1.000000000000000000, 0.000000000000000000 ) ) ;
#100434=DIRECTION ( 'NONE',  ( -0.000000000000000000, 1.000000000000000000, -0.000000000000000000 ) ) ;
#100435=CONICAL_SURFACE ( 'NONE', #52405, 0.1000000000000002554, 0.003490658503988666988 ) ;
#100436=PLANE ( 'NONE',  #2752 ) ;
#100437=EDGE_CURVE ( 'NONE', #13897, #21869, #34895, .T. ) ;
#100438=ORIENTED_EDGE ( 'NONE', *, *, #75443, .F. ) ;
#100439=EDGE_CURVE ( 'NONE', #16079, #29645, #37696, .T. ) ;
#100440=ORIENTED_EDGE ( 'NONE', *, *, #19721, .F. ) ;
#100441=EDGE_CURVE ( 'NONE', #60185, #69366, #98221, .T. ) ;
#100442=ORIENTED_EDGE ( 'NONE', *, *, #64801, .F. ) ;
#100443=CARTESIAN_POINT ( 'NONE',  ( -15.39999999999997904, 2.500000000000000000, -0.6928203230275519209 ) ) ;
#100444=CARTESIAN_POINT ( 'NONE',  ( 7.899999999999924860, 12.50000000000000000, -4.330127018922201643 ) ) ;
#100445=CARTESIAN_POINT ( 'NONE',  ( 7.499999999999960032, 12.50000000000000000, -2.276824562219559311E-15 ) ) ;
#100446=FACE_BOUND ( 'NONE', #14567, .T. ) ;
#100447=ORIENTED_EDGE ( 'NONE', *, *, #2687, .F. ) ;
#100448=DIRECTION ( 'NONE',  ( 0.000000000000000000, 0.000000000000000000, -1.000000000000000000 ) ) ;
#100449=DIRECTION ( 'NONE',  ( -0.000000000000000000, 1.000000000000000000, -0.000000000000000000 ) ) ;
#100450=ORIENTED_EDGE ( 'NONE', *, *, #119343, .T. ) ;
#100451=ADVANCED_FACE ( 'NONE', ( #4107 ), #121208, .T. ) ;
#100452=CARTESIAN_POINT ( 'NONE',  ( 15.83209681635555910, -1.499999999999999556, -5.404881881984147540 ) ) ;
#100453=DIRECTION ( 'NONE',  ( -4.274815082592931898E-19, -0.9999939076577903929, -0.003490651415223739937 ) ) ;
#100455=DIRECTION ( 'NONE',  ( 0.000000000000000000, 0.000000000000000000, -1.000000000000000000 ) ) ;
#100456=DIRECTION ( 'NONE',  ( 0.000000000000000000, 1.000000000000000000, 0.000000000000000000 ) ) ;
#100457=DIRECTION ( 'NONE',  ( 0.000000000000000000, 1.000000000000000000, 0.000000000000000000 ) ) ;
#100458=AXIS2_PLACEMENT_3D ( 'NONE', #6951, #44321, #66536 ) ;
#100459=DIRECTION ( 'NONE',  ( 0.000000000000000000, 0.000000000000000000, 1.000000000000000000 ) ) ;
#100460=FACE_OUTER_BOUND ( 'NONE', #68395, .T. ) ;
#100461=AXIS2_PLACEMENT_3D ( 'NONE', #56453, #18469, #115354 ) ;
#100462=ORIENTED_EDGE ( 'NONE', *, *, #40411, .T. ) ;
#100463=EDGE_LOOP ( 'NONE', ( #119702, #36674 ) ) ;
#100464=ORIENTED_EDGE ( 'NONE', *, *, #3427, .F. ) ;
#100465=ORIENTED_EDGE ( 'NONE', *, *, #61078, .T. ) ;
#100466=DIRECTION ( 'NONE',  ( 0.000000000000000000, 1.000000000000000000, 0.000000000000000000 ) ) ;
#100467=CARTESIAN_POINT ( 'NONE',  ( 0.8499999999999557909, 2.500000000000000000, -6.395190528383301931 ) ) ;
#100468=ORIENTED_EDGE ( 'NONE', *, *, #46480, .F. ) ;
#100469=FACE_BOUND ( 'NONE', #96579, .T. ) ;
#100470=EDGE_CURVE ( 'NONE', #34681, #76856, #83664, .T. ) ;
#100471=CARTESIAN_POINT ( 'NONE',  ( 9.599999999999914380, 2.500000000000000000, 4.330127018922196314 ) ) ;
#100472=FACE_OUTER_BOUND ( 'NONE', #61466, .T. ) ;
#100473=CARTESIAN_POINT ( 'NONE',  ( 4.149999999999938183, 2.500000000000000000, 2.165063509461097713 ) ) ;
#100474=DIRECTION ( 'NONE',  ( 0.000000000000000000, 1.000000000000000000, 0.000000000000000000 ) ) ;
#100475=DIRECTION ( 'NONE',  ( 0.000000000000000000, 1.000000000000000000, 0.000000000000000000 ) ) ;
#100476=CARTESIAN_POINT ( 'NONE',  ( -11.25000000000000178, 12.50000000000000000, -1.537336459617583584 ) ) ;
#100477=DIRECTION ( 'NONE',  ( -0.000000000000000000, -1.000000000000000000, -0.000000000000000000 ) ) ;
#100478=FACE_OUTER_BOUND ( 'NONE', #28669, .T. ) ;
#100479=VERTEX_POINT ( 'NONE', #83959 ) ;
#100480=ORIENTED_EDGE ( 'NONE', *, *, #21353, .T. ) ;
#100481=EDGE_LOOP ( 'NONE', ( #34213, #12656 ) ) ;
#100482=ORIENTED_EDGE ( 'NONE', *, *, #114716, .F. ) ;
#100483=EDGE_CURVE ( 'NONE', #10045, #33882, #72238, .T. ) ;
#100484=VERTEX_POINT ( 'NONE', #93163 ) ;
#100485=EDGE_LOOP ( 'NONE', ( #74207, #29373, #74991, #44637 ) ) ;
#100486=DIRECTION ( 'NONE',  ( -0.000000000000000000, -1.000000000000000000, -0.000000000000000000 ) ) ;
#100487=ORIENTED_EDGE ( 'NONE', *, *, #123421, .F. ) ;
#100488=AXIS2_PLACEMENT_3D ( 'NONE', #5870, #33437, #5239 ) ;
#100489=CIRCLE ( 'NONE', #77417, 0.1000000000000002554 ) ;
#100490=FACE_OUTER_BOUND ( 'NONE', #59909, .T. ) ;
#100492=DIRECTION ( 'NONE',  ( 0.000000000000000000, 0.000000000000000000, 1.000000000000000000 ) ) ;
#100493=DIRECTION ( 'NONE',  ( 0.000000000000000000, -0.9999939076577903929, 0.003490651415223739937 ) ) ;
#100494=EDGE_CURVE ( 'NONE', #39770, #6418, #14572, .T. ) ;
#100495=ORIENTED_EDGE ( 'NONE', *, *, #127895, .T. ) ;
#100496=DIRECTION ( 'NONE',  ( 0.000000000000000000, 1.000000000000000000, 0.000000000000000000 ) ) ;
#100497=AXIS2_PLACEMENT_3D ( 'NONE', #29923, #40396, #20099 ) ;
#100498=ORIENTED_EDGE ( 'NONE', *, *, #46641, .F. ) ;
#100499=VERTEX_POINT ( 'NONE', #32326 ) ;
#100500=CARTESIAN_POINT ( 'NONE',  ( -4.150000000000027889, 12.50000000000000000, -6.495190528383302464 ) ) ;
#100501=CARTESIAN_POINT ( 'NONE',  ( 6.049999999999934097, 12.50000000000000000, -2.446380397790840266 ) ) ;
#100502=DIRECTION ( 'NONE',  ( 0.000000000000000000, 1.000000000000000000, 0.000000000000000000 ) ) ;
#100503=ADVANCED_FACE ( 'NONE', ( #52575 ), #113433, .T. ) ;
#100504=EDGE_LOOP ( 'NONE', ( #47100, #40662, #115163, #37356 ) ) ;
#100505=EDGE_LOOP ( 'NONE', ( #47688, #4104 ) ) ;
#100506=CIRCLE ( 'NONE', #69198, 0.1000000000000000056 ) ;
#100507=CARTESIAN_POINT ( 'NONE',  ( -1.650000000000035660, 2.500000000000000000, 2.757883832488649656 ) ) ;
#100508=AXIS2_PLACEMENT_3D ( 'NONE', #11563, #10289, #72435 ) ;
#100509=DIRECTION ( 'NONE',  ( 0.000000000000000000, 1.000000000000000000, 0.000000000000000000 ) ) ;
#100510=FACE_OUTER_BOUND ( 'NONE', #9555, .T. ) ;
#100511=CARTESIAN_POINT ( 'NONE',  ( -5.200000000000024158, 12.50000000000000000, -4.676537180435977881 ) ) ;
#100512=EDGE_LOOP ( 'NONE', ( #88299, #68441, #67442, #88502 ) ) ;
#100513=DIRECTION ( 'NONE',  ( -0.000000000000000000, -1.000000000000000000, -0.000000000000000000 ) ) ;
#100514=VERTEX_POINT ( 'NONE', #53874 ) ;
#100515=CARTESIAN_POINT ( 'NONE',  ( -2.700000000000029932, 2.500000000000000000, -4.576537180435977348 ) ) ;
#100516=ORIENTED_EDGE ( 'NONE', *, *, #17635, .F. ) ;
#100517=CARTESIAN_POINT ( 'NONE',  ( 87.50000000000001421, 3.974992050023849810, 6.359987280038159163 ) ) ;
#100518=EDGE_CURVE ( 'NONE', #93018, #86595, #64774, .T. ) ;
#100519=DIRECTION ( 'NONE',  ( 0.000000000000000000, 0.000000000000000000, 1.000000000000000000 ) ) ;
#100520=AXIS2_PLACEMENT_3D ( 'NONE', #107706, #20620, #38999 ) ;
#100522=DIRECTION ( 'NONE',  ( 0.000000000000000000, 0.000000000000000000, -1.000000000000000000 ) ) ;
#100523=EDGE_LOOP ( 'NONE', ( #55962, #8801, #4196, #53572 ) ) ;
#100524=EDGE_CURVE ( 'NONE', #99397, #72027, #79470, .T. ) ;
#100525=DIRECTION ( 'NONE',  ( -0.000000000000000000, -1.000000000000000000, -0.000000000000000000 ) ) ;
#100526=LINE ( 'NONE', #82192, #44478 ) ;
#100527=ORIENTED_EDGE ( 'NONE', *, *, #83709, .T. ) ;
#100528=ORIENTED_EDGE ( 'NONE', *, *, #115026, .F. ) ;
#100529=EDGE_CURVE ( 'NONE', #5370, #50596, #33499, .T. ) ;
#100530=ADVANCED_FACE ( 'NONE', ( #64963 ), #94423, .T. ) ;
#100531=VERTEX_POINT ( 'NONE', #102960 ) ;
#100532=DIRECTION ( 'NONE',  ( 0.000000000000000000, -0.9999939076577903929, 0.003490651415223739937 ) ) ;
#100533=CARTESIAN_POINT ( 'NONE',  ( -13.14999999999999147, 2.500000000000000000, -1.818653347947323917 ) ) ;
#100534=CARTESIAN_POINT ( 'NONE',  ( 19.95908882845300170, 2.629614671951224114, 2.273431397254408903 ) ) ;
#100535=ADVANCED_FACE ( 'NONE', ( #64333 ), #46015, .T. ) ;
#100536=DIRECTION ( 'NONE',  ( 0.000000000000000000, -0.9999939076577903929, 0.003490651415223739937 ) ) ;
#100537=EDGE_CURVE ( 'NONE', #97073, #15146, #6270, .T. ) ;
#100538=DIRECTION ( 'NONE',  ( -4.274815082592931898E-19, -0.9999939076577903929, -0.003490651415223739937 ) ) ;
#100539=LINE ( 'NONE', #82201, #36096 ) ;
#100540=CARTESIAN_POINT ( 'NONE',  ( -5.850000000000018296, 2.500000000000000000, 5.802370205355744659 ) ) ;
#100541=FACE_OUTER_BOUND ( 'NONE', #104607, .T. ) ;
#100542=DIRECTION ( 'NONE',  ( 0.000000000000000000, -0.9999939076577903929, 0.003490651415223739937 ) ) ;
#100543=ADVANCED_FACE ( 'NONE', ( #92496 ), #27215, .T. ) ;
#100544=VECTOR ( 'NONE', #30198, 1000.000000000000000 ) ;
#100545=CIRCLE ( 'NONE', #121379, 0.06509327318403745899 ) ;
#100546=CONICAL_SURFACE ( 'NONE', #50373, 0.09999999999999982514, 0.003490658503988666988 ) ;
#100547=EDGE_CURVE ( 'NONE', #4391, #95241, #20959, .T. ) ;
#100548=ADVANCED_FACE ( 'NONE', ( #63046 ), #112905, .T. ) ;
#100549=CIRCLE ( 'NONE', #52532, 0.1000000000000000472 ) ;
#100550=ADVANCED_FACE ( 'NONE', ( #95086 ), #4219, .T. ) ;
#100551=ORIENTED_EDGE ( 'NONE', *, *, #25748, .F. ) ;
#100552=DIRECTION ( 'NONE',  ( 0.000000000000000000, 0.000000000000000000, 1.000000000000000000 ) ) ;
#100553=PLANE ( 'NONE',  #30763 ) ;
#100554=DIRECTION ( 'NONE',  ( -0.000000000000000000, 1.000000000000000000, -0.000000000000000000 ) ) ;
#100555=DIRECTION ( 'NONE',  ( 0.000000000000000000, 0.000000000000000000, 1.000000000000000000 ) ) ;
#100556=EDGE_CURVE ( 'NONE', #85131, #118944, #117265, .T. ) ;
#100557=ORIENTED_EDGE ( 'NONE', *, *, #100070, .T. ) ;
#100558=CARTESIAN_POINT ( 'NONE',  ( -3.950000000000026379, 2.500000000000000000, -1.818653347947326138 ) ) ;
#100559=DIRECTION ( 'NONE',  ( 0.000000000000000000, -0.000000000000000000, 1.000000000000000000 ) ) ;
#100560=CARTESIAN_POINT ( 'NONE',  ( 6.899999999999926636, 2.500000000000000000, 0.2464101615137736789 ) ) ;
#100561=ORIENTED_EDGE ( 'NONE', *, *, #2421, .T. ) ;
#100562=EDGE_LOOP ( 'NONE', ( #47509, #88886, #81624, #113171 ) ) ;
#100563=DIRECTION ( 'NONE',  ( 0.000000000000000000, 1.000000000000000000, 0.000000000000000000 ) ) ;
#100564=VECTOR ( 'NONE', #125591, 1000.000000000000000 ) ;
#100565=ORIENTED_EDGE ( 'NONE', *, *, #67555, .F. ) ;
#100566=EDGE_LOOP ( 'NONE', ( #50636, #21144, #86585, #84016 ) ) ;
#100567=DIRECTION ( 'NONE',  ( 0.000000000000000000, 0.000000000000000000, 1.000000000000000000 ) ) ;
#100568=CARTESIAN_POINT ( 'NONE',  ( 18.78720903128162334, 2.539625591035298946, -4.564429507521253093 ) ) ;
#100569=CARTESIAN_POINT ( 'NONE',  ( 12.49999999999993960, 12.50000000000000000, 4.330127018922196314 ) ) ;
#100570=DIRECTION ( 'NONE',  ( 0.000000000000000000, 1.000000000000000000, 0.000000000000000000 ) ) ;
#100571=AXIS2_PLACEMENT_3D ( 'NONE', #115169, #65444, #15691 ) ;
#100572=EDGE_LOOP ( 'NONE', ( #17743, #66834 ) ) ;
#100573=VECTOR ( 'NONE', #98568, 1000.000000000000000 ) ;
#100574=CARTESIAN_POINT ( 'NONE',  ( 0.000000000000000000, 12.50000000000000000, 0.000000000000000000 ) ) ;
#100575=VERTEX_POINT ( 'NONE', #36819 ) ;
#100577=CARTESIAN_POINT ( 'NONE',  ( 16.56576425165006583, -1.500000000000000666, 6.084390597445813675 ) ) ;
#100579=ORIENTED_EDGE ( 'NONE', *, *, #30011, .F. ) ;
#100580=AXIS2_PLACEMENT_3D ( 'NONE', #39388, #79296, #119207 ) ;
#100581=EDGE_CURVE ( 'NONE', #82804, #94907, #37610, .T. ) ;
#100582=ORIENTED_EDGE ( 'NONE', *, *, #53653, .F. ) ;
#100583=ORIENTED_EDGE ( 'NONE', *, *, #53993, .F. ) ;
#100584=EDGE_CURVE ( 'NONE', #18587, #71296, #31351, .T. ) ;
#100585=ORIENTED_EDGE ( 'NONE', *, *, #70945, .T. ) ;
#100586=CARTESIAN_POINT ( 'NONE',  ( 9.149999999999918643, 12.50000000000000000, 2.165063509461097713 ) ) ;
#100587=CARTESIAN_POINT ( 'NONE',  ( 10.63722763381497849, 2.499999999999999556, 8.014330155767298791 ) ) ;
#100588=FACE_OUTER_BOUND ( 'NONE', #30819, .T. ) ;
#100589=FACE_BOUND ( 'NONE', #100036, .T. ) ;
#100590=DIRECTION ( 'NONE',  ( 0.000000000000000000, 0.000000000000000000, 1.000000000000000000 ) ) ;
#100592=CARTESIAN_POINT ( 'NONE',  ( 9.199999999999915801, 2.500000000000000000, -4.430127018922202176 ) ) ;
#100593=DIRECTION ( 'NONE',  ( 0.000000000000000000, 0.000000000000000000, 1.000000000000000000 ) ) ;
#100594=AXIS2_PLACEMENT_3D ( 'NONE', #128113, #19429, #10272 ) ;
#100595=EDGE_CURVE ( 'NONE', #104576, #76747, #75245, .T. ) ;
#100596=AXIS2_PLACEMENT_3D ( 'NONE', #101737, #120093, #30439 ) ;
#100597=CARTESIAN_POINT ( 'NONE',  ( -9.600000000000008527, 12.50000000000000000, -3.702399969078682851 ) ) ;
#100598=FACE_OUTER_BOUND ( 'NONE', #59413, .T. ) ;
#100599=DIRECTION ( 'NONE',  ( -0.000000000000000000, 1.000000000000000000, -0.000000000000000000 ) ) ;
#100600=AXIS2_PLACEMENT_3D ( 'NONE', #43003, #1741, #111038 ) ;
#100601=DIRECTION ( 'NONE',  ( -0.000000000000000000, 1.000000000000000000, -0.000000000000000000 ) ) ;
#100602=ORIENTED_EDGE ( 'NONE', *, *, #72546, .T. ) ;
#100603=AXIS2_PLACEMENT_3D ( 'NONE', #9992, #89833, #87246 ) ;
#100604=ORIENTED_EDGE ( 'NONE', *, *, #43805, .F. ) ;
#100605=VERTEX_POINT ( 'NONE', #117933 ) ;
#100606=ORIENTED_EDGE ( 'NONE', *, *, #10657, .T. ) ;
#100608=CARTESIAN_POINT ( 'NONE',  ( -2.500000000000030642, 2.500000000000000000, -5.022947341949754119 ) ) ;
#100609=ORIENTED_EDGE ( 'NONE', *, *, #107902, .F. ) ;
#100610=FACE_BOUND ( 'NONE', #53970, .T. ) ;
#100611=DIRECTION ( 'NONE',  ( 0.000000000000000000, 1.000000000000000000, 0.000000000000000000 ) ) ;
#100612=ORIENTED_EDGE ( 'NONE', *, *, #71009, .F. ) ;
#100613=DIRECTION ( 'NONE',  ( -4.274815082592931898E-19, -0.9999939076577903929, -0.003490651415223739937 ) ) ;
#100614=CARTESIAN_POINT ( 'NONE',  ( -11.89999999999999503, 2.500000000000000000, 4.676537180435972552 ) ) ;
#100615=FACE_OUTER_BOUND ( 'NONE', #74945, .T. ) ;
#100616=DIRECTION ( 'NONE',  ( -0.000000000000000000, -1.000000000000000000, -0.000000000000000000 ) ) ;
#100617=ORIENTED_EDGE ( 'NONE', *, *, #103965, .T. ) ;
#100618=CARTESIAN_POINT ( 'NONE',  ( 9.199999999999915801, 2.500000000000000000, -4.230127018922201998 ) ) ;
#100619=ADVANCED_FACE ( 'NONE', ( #66897 ), #85261, .T. ) ;
#100620=ORIENTED_EDGE ( 'NONE', *, *, #47474, .T. ) ;
#100621=CONICAL_SURFACE ( 'NONE', #44196, 0.09999999999999982514, 0.003490658503988666988 ) ;
#100622=EDGE_LOOP ( 'NONE', ( #19652, #3312, #62795, #57814 ) ) ;
#100623=DIRECTION ( 'NONE',  ( 0.000000000000000000, 0.000000000000000000, 1.000000000000000000 ) ) ;
#100624=AXIS2_PLACEMENT_3D ( 'NONE', #64453, #3607, #104385 ) ;
#100625=DIRECTION ( 'NONE',  ( 0.000000000000000000, 1.000000000000000000, 0.000000000000000000 ) ) ;
#100626=ORIENTED_EDGE ( 'NONE', *, *, #79081, .F. ) ;
#100627=DIRECTION ( 'NONE',  ( 0.000000000000000000, 1.000000000000000000, 0.000000000000000000 ) ) ;
#100628=CARTESIAN_POINT ( 'NONE',  ( -7.300000000000018474, 2.500000000000000000, -3.983716857408426293 ) ) ;
#100629=CIRCLE ( 'NONE', #117328, 0.06509327318403745899 ) ;
#100630=DIRECTION ( 'NONE',  ( -0.000000000000000000, -1.000000000000000000, -0.000000000000000000 ) ) ;
#100631=VECTOR ( 'NONE', #98545, 1000.000000000000000 ) ;
#100632=DIRECTION ( 'NONE',  ( 0.000000000000000000, 0.000000000000000000, 1.000000000000000000 ) ) ;
#100633=ORIENTED_EDGE ( 'NONE', *, *, #126097, .F. ) ;
#100634=CONICAL_SURFACE ( 'NONE', #19060, 0.1000000000000002554, 0.003490658503988666988 ) ;
#100635=EDGE_CURVE ( 'NONE', #25412, #64421, #75429, .T. ) ;
#100636=EDGE_CURVE ( 'NONE', #57597, #66863, #35553, .T. ) ;
#100637=DIRECTION ( 'NONE',  ( -0.000000000000000000, -1.000000000000000000, -0.000000000000000000 ) ) ;
#100638=ORIENTED_EDGE ( 'NONE', *, *, #99814, .T. ) ;
#100639=DIRECTION ( 'NONE',  ( 0.000000000000000000, 1.000000000000000000, 0.000000000000000000 ) ) ;
#100640=EDGE_LOOP ( 'NONE', ( #10681, #68197, #4392, #67115 ) ) ;
#100641=DIRECTION ( 'NONE',  ( -0.000000000000000000, 1.000000000000000000, -0.000000000000000000 ) ) ;
#100642=EDGE_LOOP ( 'NONE', ( #112431, #27969, #1227, #78824 ) ) ;
#100643=FACE_OUTER_BOUND ( 'NONE', #25786, .T. ) ;
#100644=DIRECTION ( 'NONE',  ( 0.000000000000000000, 0.000000000000000000, -1.000000000000000000 ) ) ;
#100645=DIRECTION ( 'NONE',  ( 0.000000000000000000, 1.000000000000000000, 0.000000000000000000 ) ) ;
#100646=LINE ( 'NONE', #111099, #11115 ) ;
#100647=EDGE_CURVE ( 'NONE', #89951, #17587, #105554, .T. ) ;
#100648=FACE_OUTER_BOUND ( 'NONE', #123619, .T. ) ;
#100649=ORIENTED_EDGE ( 'NONE', *, *, #8198, .F. ) ;
#100650=ORIENTED_EDGE ( 'NONE', *, *, #31802, .T. ) ;
#100651=ORIENTED_EDGE ( 'NONE', *, *, #117105, .T. ) ;
#100652=FACE_OUTER_BOUND ( 'NONE', #1773, .T. ) ;
#100653=CARTESIAN_POINT ( 'NONE',  ( 14.79999999999989235, 2.500000000000000000, 0.2464101615137735679 ) ) ;
#100654=FACE_OUTER_BOUND ( 'NONE', #96715, .T. ) ;
#100655=ORIENTED_EDGE ( 'NONE', *, *, #68965, .T. ) ;
#100656=ORIENTED_EDGE ( 'NONE', *, *, #58889, .T. ) ;
#100657=EDGE_LOOP ( 'NONE', ( #24289, #97951, #47478, #113724 ) ) ;
#100658=CARTESIAN_POINT ( 'NONE',  ( 4.799999999999935874, 12.50000000000000000, 0.3464101615137735735 ) ) ;
#100659=CONICAL_SURFACE ( 'NONE', #67188, 0.1000000000000000472, 0.003490658503988666988 ) ;
#100660=ORIENTED_EDGE ( 'NONE', *, *, #39862, .F. ) ;
#100661=CARTESIAN_POINT ( 'NONE',  ( 7.499999999999927169, 2.500000000000000000, 3.537306695894645081 ) ) ;
#100662=CONICAL_SURFACE ( 'NONE', #63027, 0.1000000000000000472, 0.003490658503988666988 ) ;
#100663=PLANE ( 'NONE',  #120068 ) ;
#100664=CARTESIAN_POINT ( 'NONE',  ( 2.499999999999947153, 2.500000000000000000, -3.537306695894649966 ) ) ;
#100665=LINE ( 'NONE', #69940, #17229 ) ;
#100666=DIRECTION ( 'NONE',  ( 0.000000000000000000, -0.9999939076577903929, 0.003490651415223739937 ) ) ;
#100667=DIRECTION ( 'NONE',  ( -0.000000000000000000, 1.000000000000000000, -0.000000000000000000 ) ) ;
#100668=DIRECTION ( 'NONE',  ( 0.000000000000000000, 1.000000000000000000, 0.000000000000000000 ) ) ;
#100669=AXIS2_PLACEMENT_3D ( 'NONE', #50357, #80485, #120393 ) ;
#100670=ORIENTED_EDGE ( 'NONE', *, *, #56087, .F. ) ;
#100671=CIRCLE ( 'NONE', #75539, 0.06509327318403745899 ) ;
#100672=EDGE_LOOP ( 'NONE', ( #44184, #126579, #129444, #87475 ) ) ;
#100673=EDGE_CURVE ( 'NONE', #59628, #77485, #39767, .T. ) ;
#100674=LINE ( 'NONE', #11003, #25737 ) ;
#100675=CONICAL_SURFACE ( 'NONE', #54692, 0.1000000000000000472, 0.003490658503988666988 ) ;
#100676=DIRECTION ( 'NONE',  ( 0.000000000000000000, 1.000000000000000000, 0.000000000000000000 ) ) ;
#100677=VERTEX_POINT ( 'NONE', #115337 ) ;
#100678=ORIENTED_EDGE ( 'NONE', *, *, #108921, .T. ) ;
#100679=ADVANCED_FACE ( 'NONE', ( #65615 ), #52269, .T. ) ;
#100681=DIRECTION ( 'NONE',  ( 0.000000000000000000, 0.000000000000000000, 1.000000000000000000 ) ) ;
#100682=DIRECTION ( 'NONE',  ( 0.000000000000000000, -0.000000000000000000, 1.000000000000000000 ) ) ;
#100684=AXIS2_PLACEMENT_3D ( 'NONE', #92697, #33144, #73060 ) ;
#100685=CARTESIAN_POINT ( 'NONE',  ( 1.249999999999988454, 2.500000000000000000, 2.065063509461097624 ) ) ;
#100686=DIRECTION ( 'NONE',  ( -4.274815082592931898E-19, -0.9999939076577903929, -0.003490651415223739937 ) ) ;
#100687=FACE_OUTER_BOUND ( 'NONE', #128374, .T. ) ;
#100688=DIRECTION ( 'NONE',  ( 0.000000000000000000, -0.000000000000000000, 1.000000000000000000 ) ) ;
#100689=VECTOR ( 'NONE', #12807, 1000.000000000000000 ) ;
#100690=DIRECTION ( 'NONE',  ( -4.274815082592931898E-19, -0.9999939076577903929, -0.003490651415223739937 ) ) ;
#100691=EDGE_CURVE ( 'NONE', #4868, #11053, #12537, .T. ) ;
#100692=EDGE_CURVE ( 'NONE', #37929, #56654, #102444, .T. ) ;
#100693=EDGE_CURVE ( 'NONE', #109444, #16630, #119157, .T. ) ;
#100694=VECTOR ( 'NONE', #67761, 1000.000000000000000 ) ;
#100695=DIRECTION ( 'NONE',  ( 0.000000000000000000, 0.000000000000000000, 1.000000000000000000 ) ) ;
#100696=ORIENTED_EDGE ( 'NONE', *, *, #55447, .T. ) ;
#100697=ORIENTED_EDGE ( 'NONE', *, *, #33018, .F. ) ;
#100698=EDGE_CURVE ( 'NONE', #127171, #27644, #94120, .T. ) ;
#100699=AXIS2_PLACEMENT_3D ( 'NONE', #35441, #16400, #26901 ) ;
#100700=VERTEX_POINT ( 'NONE', #17797 ) ;
#100701=ORIENTED_EDGE ( 'NONE', *, *, #65683, .F. ) ;
#100702=EDGE_LOOP ( 'NONE', ( #44294, #32074 ) ) ;
#100703=DIRECTION ( 'NONE',  ( 0.000000000000000000, 0.000000000000000000, 1.000000000000000000 ) ) ;
#100705=ADVANCED_FACE ( 'NONE', ( #6040 ), #77113, .T. ) ;
#100706=EDGE_LOOP ( 'NONE', ( #50602, #22030, #4979, #115040 ) ) ;
#100707=LINE ( 'NONE', #79168, #29826 ) ;
#100709=CARTESIAN_POINT ( 'NONE',  ( -14.39999999999998614, 12.50000000000000000, 0.3464101615137758494 ) ) ;
#100710=CARTESIAN_POINT ( 'NONE',  ( -8.100000000000010303, 12.50000000000000000, 4.611443907251934426 ) ) ;
#100711=ORIENTED_EDGE ( 'NONE', *, *, #3997, .F. ) ;
#100712=DIRECTION ( 'NONE',  ( -0.000000000000000000, 1.000000000000000000, -0.000000000000000000 ) ) ;
#100713=DIRECTION ( 'NONE',  ( 0.000000000000000000, 0.000000000000000000, -1.000000000000000000 ) ) ;
#100715=ORIENTED_EDGE ( 'NONE', *, *, #47438, .F. ) ;
#100716=ORIENTED_EDGE ( 'NONE', *, *, #107308, .T. ) ;
#100717=CIRCLE ( 'NONE', #10816, 0.06509327318403745899 ) ;
#100718=VERTEX_POINT ( 'NONE', #15203 ) ;
#100719=FACE_OUTER_BOUND ( 'NONE', #56037, .T. ) ;
#100720=CONICAL_SURFACE ( 'NONE', #61015, 0.1000000000000000472, 0.003490658503988666988 ) ;
#100721=AXIS2_PLACEMENT_3D ( 'NONE', #60470, #111466, #19883 ) ;
#100722=LINE ( 'NONE', #119721, #61338 ) ;
#100723=CARTESIAN_POINT ( 'NONE',  ( 1.849999999999949685, 2.500000000000000000, 1.918653347947321564 ) ) ;
#100724=AXIS2_PLACEMENT_3D ( 'NONE', #93835, #14603, #44085 ) ;
#100725=CARTESIAN_POINT ( 'NONE',  ( 4.149999999999939959, 2.500000000000000000, -6.595190528383302109 ) ) ;
#100726=AXIS2_PLACEMENT_3D ( 'NONE', #61870, #102429, #70388 ) ;
#100727=ORIENTED_EDGE ( 'NONE', *, *, #108506, .F. ) ;
#100728=CARTESIAN_POINT ( 'NONE',  ( 9.599999999999914380, 12.50000000000000000, -3.702399969078687292 ) ) ;
#100729=FACE_OUTER_BOUND ( 'NONE', #57598, .T. ) ;
#100730=CARTESIAN_POINT ( 'NONE',  ( -11.84999999999999609, 12.50000000000000000, 2.511473670974873507 ) ) ;
#100731=DIRECTION ( 'NONE',  ( 0.000000000000000000, 1.000000000000000000, 0.000000000000000000 ) ) ;
#100732=AXIS2_PLACEMENT_3D ( 'NONE', #14781, #54728, #94656 ) ;
#100733=EDGE_LOOP ( 'NONE', ( #27991, #110308, #65743, #12202 ) ) ;
#100734=EDGE_CURVE ( 'NONE', #61946, #19850, #45995, .T. ) ;
#100735=VERTEX_POINT ( 'NONE', #9281 ) ;
#100736=ORIENTED_EDGE ( 'NONE', *, *, #119899, .F. ) ;
#100737=LINE ( 'NONE', #102050, #72775 ) ;
#100738=DIRECTION ( 'NONE',  ( 0.000000000000000000, -0.9999939076577903929, 0.003490651415223739937 ) ) ;
#100739=FACE_BOUND ( 'NONE', #75450, .T. ) ;
#100741=CARTESIAN_POINT ( 'NONE',  ( 3.349999999999943689, 2.500000000000000000, 2.265063509461097357 ) ) ;
#100742=FACE_OUTER_BOUND ( 'NONE', #53152, .T. ) ;
#100743=EDGE_CURVE ( 'NONE', #112572, #44266, #19074, .T. ) ;
#100744=DIRECTION ( 'NONE',  ( 0.000000000000000000, 0.000000000000000000, 1.000000000000000000 ) ) ;
#100745=DIRECTION ( 'NONE',  ( 0.000000000000000000, 1.000000000000000000, 0.000000000000000000 ) ) ;
#100746=DIRECTION ( 'NONE',  ( 0.000000000000000000, 0.000000000000000000, 1.000000000000000000 ) ) ;
#100747=ORIENTED_EDGE ( 'NONE', *, *, #86199, .F. ) ;
#100748=AXIS2_PLACEMENT_3D ( 'NONE', #67869, #65936, #128094 ) ;
#100749=DIRECTION ( 'NONE',  ( 0.000000000000000000, 1.000000000000000000, 0.000000000000000000 ) ) ;
#100750=CARTESIAN_POINT ( 'NONE',  ( -3.150000000000029221, 2.500000000000000000, 2.611473670974873151 ) ) ;
#100751=VERTEX_POINT ( 'NONE', #59027 ) ;
#100752=ORIENTED_EDGE ( 'NONE', *, *, #46817, .T. ) ;
#100753=DIRECTION ( 'NONE',  ( 0.000000000000000000, 0.000000000000000000, 1.000000000000000000 ) ) ;
#100754=DIRECTION ( 'NONE',  ( 0.000000000000000000, 1.000000000000000000, 0.000000000000000000 ) ) ;
#100755=FACE_BOUND ( 'NONE', #2460, .T. ) ;
#100756=CIRCLE ( 'NONE', #8813, 0.06509327318403745899 ) ;
#100757=FACE_OUTER_BOUND ( 'NONE', #56754, .T. ) ;
#100758=CIRCLE ( 'NONE', #56834, 0.09999999999999982514 ) ;
#100759=VECTOR ( 'NONE', #13921, 1000.000000000000000 ) ;
#100760=CIRCLE ( 'NONE', #67293, 0.06509327318403745899 ) ;
#100761=DIRECTION ( 'NONE',  ( -0.000000000000000000, 1.000000000000000000, -0.000000000000000000 ) ) ;
#100762=VERTEX_POINT ( 'NONE', #58397 ) ;
#100763=DIRECTION ( 'NONE',  ( 0.000000000000000000, -0.9999939076577903929, 0.003490651415223739937 ) ) ;
#100764=DIRECTION ( 'NONE',  ( 0.000000000000000000, 1.000000000000000000, 0.000000000000000000 ) ) ;
#100765=ORIENTED_EDGE ( 'NONE', *, *, #66567, .T. ) ;
#100766=AXIS2_PLACEMENT_3D ( 'NONE', #110880, #113299, #124422 ) ;
#100767=DIRECTION ( 'NONE',  ( 0.000000000000000000, 1.000000000000000000, 0.000000000000000000 ) ) ;
#100768=DIRECTION ( 'NONE',  ( 0.000000000000000000, 0.000000000000000000, -1.000000000000000000 ) ) ;
#100769=ADVANCED_FACE ( 'NONE', ( #48566 ), #70851, .T. ) ;
#100770=CIRCLE ( 'NONE', #104889, 0.06509327318403745899 ) ;
#100771=AXIS2_PLACEMENT_3D ( 'NONE', #36791, #117896, #107443 ) ;
#100772=AXIS2_PLACEMENT_3D ( 'NONE', #68773, #109345, #29506 ) ;
#100773=CARTESIAN_POINT ( 'NONE',  ( -8.750000000000010658, 2.500000000000000000, -7.188010851410848723 ) ) ;
#100775=AXIS2_PLACEMENT_3D ( 'NONE', #70669, #19647, #631 ) ;
#100776=EDGE_CURVE ( 'NONE', #111375, #36539, #69474, .T. ) ;
#100777=EDGE_LOOP ( 'NONE', ( #1821, #26117 ) ) ;
#100778=CARTESIAN_POINT ( 'NONE',  ( 4.999999999999969802, 2.500000000000000000, 4.230127018922196669 ) ) ;
#100779=CIRCLE ( 'NONE', #94535, 0.06509327318403745899 ) ;
#100780=CARTESIAN_POINT ( 'NONE',  ( -8.150000000000014566, 2.500000000000000000, -6.148780366869520897 ) ) ;
#100781=CARTESIAN_POINT ( 'NONE',  ( 6.249999999999967137, 12.50000000000000000, -2.165063509461101710 ) ) ;
#100782=VERTEX_POINT ( 'NONE', #98949 ) ;
#100783=EDGE_CURVE ( 'NONE', #7958, #46669, #72910, .T. ) ;
#100784=ORIENTED_EDGE ( 'NONE', *, *, #21025, .T. ) ;
#100785=ADVANCED_FACE ( 'NONE', ( #89127 ), #43688, .T. ) ;
#100786=CARTESIAN_POINT ( 'NONE',  ( -8.300000000000011369, 12.50000000000000000, -2.276824562219559311E-15 ) ) ;
#100787=EDGE_LOOP ( 'NONE', ( #4822, #28527, #66636, #15007 ) ) ;
#100788=CARTESIAN_POINT ( 'NONE',  ( -1.050000000000038680, 12.50000000000000000, 2.446380397790835826 ) ) ;
#100789=CARTESIAN_POINT ( 'NONE',  ( 0.5999999999999547917, 2.500000000000000000, 3.983716857408420076 ) ) ;
#100791=ORIENTED_EDGE ( 'NONE', *, *, #57497, .T. ) ;
#100792=ADVANCED_FACE ( 'NONE', ( #81248 ), #88469, .T. ) ;
#100793=LINE ( 'NONE', #3894, #1507 ) ;
#100794=DIRECTION ( 'NONE',  ( -0.000000000000000000, 1.000000000000000000, -0.000000000000000000 ) ) ;
#100795=CARTESIAN_POINT ( 'NONE',  ( 9.399999999999915090, 2.500000000000000000, 4.576537180435972019 ) ) ;
#100796=DIRECTION ( 'NONE',  ( -0.000000000000000000, -1.000000000000000000, -0.000000000000000000 ) ) ;
#100797=DIRECTION ( 'NONE',  ( 0.000000000000000000, 0.000000000000000000, -1.000000000000000000 ) ) ;
#100798=ADVANCED_FACE ( 'NONE', ( #128435 ), #28934, .T. ) ;
#100799=CARTESIAN_POINT ( 'NONE',  ( -8.550000000000013145, 12.50000000000000000, -6.841600689897073373 ) ) ;
#100800=ORIENTED_EDGE ( 'NONE', *, *, #67572, .T. ) ;
#100801=ORIENTED_EDGE ( 'NONE', *, *, #87201, .F. ) ;
#100802=DIRECTION ( 'NONE',  ( -4.274815082592931898E-19, -0.9999939076577903929, -0.003490651415223739937 ) ) ;
#100803=ORIENTED_EDGE ( 'NONE', *, *, #68865, .T. ) ;
#100804=CIRCLE ( 'NONE', #75671, 0.1000000000000002554 ) ;
#100806=VECTOR ( 'NONE', #21048, 1000.000000000000000 ) ;
#100807=CIRCLE ( 'NONE', #452, 0.1000000000000002554 ) ;
#100808=ORIENTED_EDGE ( 'NONE', *, *, #113504, .T. ) ;
#100809=EDGE_LOOP ( 'NONE', ( #85554, #5981 ) ) ;
#100810=VERTEX_POINT ( 'NONE', #110062 ) ;
#100811=DIRECTION ( 'NONE',  ( 0.000000000000000000, 1.000000000000000000, 0.000000000000000000 ) ) ;
#100812=CARTESIAN_POINT ( 'NONE',  ( 7.699999999999922018, 12.50000000000000000, 0.3464101615137735735 ) ) ;
#100813=VECTOR ( 'NONE', #72706, 1000.000000000000000 ) ;
#100814=CARTESIAN_POINT ( 'NONE',  ( 3.949999999999940670, 12.50000000000000000, 1.753560074763284016 ) ) ;
#100815=CIRCLE ( 'NONE', #102866, 0.09999999999999999167 ) ;
#100817=CARTESIAN_POINT ( 'NONE',  ( 7.049999999999928768, 12.50000000000000000, 6.430097255199259010 ) ) ;
#100818=CARTESIAN_POINT ( 'NONE',  ( -9.350000000000006750, 12.50000000000000000, 1.753560074763284016 ) ) ;
#100819=DIRECTION ( 'NONE',  ( 0.000000000000000000, 0.000000000000000000, 1.000000000000000000 ) ) ;
#100820=AXIS2_PLACEMENT_3D ( 'NONE', #53972, #53340, #73597 ) ;
#100821=DIRECTION ( 'NONE',  ( 0.000000000000000000, 0.000000000000000000, 1.000000000000000000 ) ) ;
#100822=LINE ( 'NONE', #28890, #109308 ) ;
#100823=AXIS2_PLACEMENT_3D ( 'NONE', #119035, #107917, #58195 ) ;
#100824=DIRECTION ( 'NONE',  ( 0.000000000000000000, 0.000000000000000000, 1.000000000000000000 ) ) ;
#100825=VECTOR ( 'NONE', #1846, 1000.000000000000000 ) ;
#100826=ORIENTED_EDGE ( 'NONE', *, *, #115570, .T. ) ;
#100827=EDGE_CURVE ( 'NONE', #119283, #109616, #95986, .T. ) ;
#100828=DIRECTION ( 'NONE',  ( 0.000000000000000000, 0.000000000000000000, 1.000000000000000000 ) ) ;
#100829=ORIENTED_EDGE ( 'NONE', *, *, #650, .T. ) ;
#100830=VERTEX_POINT ( 'NONE', #109408 ) ;
#100831=LINE ( 'NONE', #121134, #73349 ) ;
#100832=CARTESIAN_POINT ( 'NONE',  ( -4.600000000000025402, 2.500000000000000000, 4.230127018922196669 ) ) ;
#100833=ADVANCED_FACE ( 'NONE', ( #121163 ), #37418, .T. ) ;
#100834=AXIS2_PLACEMENT_3D ( 'NONE', #56760, #96695, #86885 ) ;
#100835=FACE_OUTER_BOUND ( 'NONE', #86552, .T. ) ;
#100836=CARTESIAN_POINT ( 'NONE',  ( 6.249999999999968914, 12.50000000000000000, -6.495190528383302464 ) ) ;
#100837=DIRECTION ( 'NONE',  ( 0.000000000000000000, 0.000000000000000000, -1.000000000000000000 ) ) ;
#100838=DIRECTION ( 'NONE',  ( -4.274815082592931898E-19, -0.9999939076577903929, -0.003490651415223739937 ) ) ;
#100839=VERTEX_POINT ( 'NONE', #9921 ) ;
#100840=ADVANCED_FACE ( 'NONE', ( #60334 ), #31164, .T. ) ;
#100841=ADVANCED_FACE ( 'NONE', ( #30230 ), #112714, .T. ) ;
#100842=EDGE_CURVE ( 'NONE', #108104, #79172, #91775, .T. ) ;
#100843=CIRCLE ( 'NONE', #36020, 0.06509327318403745899 ) ;
#100844=VERTEX_POINT ( 'NONE', #30872 ) ;
#100845=CARTESIAN_POINT ( 'NONE',  ( 13.34999999999990017, 2.500000000000000000, 2.165063509461097713 ) ) ;
#100846=CIRCLE ( 'NONE', #128056, 0.06509327318403745899 ) ;
#100847=EDGE_LOOP ( 'NONE', ( #129469, #50699, #87184, #13387 ) ) ;
#100848=DIRECTION ( 'NONE',  ( 0.000000000000000000, 1.000000000000000000, 0.000000000000000000 ) ) ;
#100849=ADVANCED_FACE ( 'NONE', ( #10547 ), #116809, .T. ) ;
#100850=EDGE_LOOP ( 'NONE', ( #56872, #2637 ) ) ;
#100851=VERTEX_POINT ( 'NONE', #100866 ) ;
#100852=AXIS2_PLACEMENT_3D ( 'NONE', #19278, #79517, #119414 ) ;
#100854=CARTESIAN_POINT ( 'NONE',  ( 6.649999999999931966, 2.500000000000000000, -5.802370205355749988 ) ) ;
#100855=CIRCLE ( 'NONE', #98702, 0.06509327318403745899 ) ;
#100856=EDGE_CURVE ( 'NONE', #850, #116295, #51151, .T. ) ;
#100857=CIRCLE ( 'NONE', #2650, 0.09999999999999999167 ) ;
#100858=ADVANCED_FACE ( 'NONE', ( #108116 ), #121024, .T. ) ;
#100859=CARTESIAN_POINT ( 'NONE',  ( -13.29999999999999005, 12.50000000000000000, -4.330127018922198978 ) ) ;
#100860=CONICAL_SURFACE ( 'NONE', #90388, 0.1000000000000000056, 0.003490658503988666988 ) ;
#100861=DIRECTION ( 'NONE',  ( 0.000000000000000000, 0.000000000000000000, 1.000000000000000000 ) ) ;
#100862=LINE ( 'NONE', #120521, #20018 ) ;
#100863=EDGE_LOOP ( 'NONE', ( #57301, #116377 ) ) ;
#100864=DIRECTION ( 'NONE',  ( -0.000000000000000000, 1.000000000000000000, -0.000000000000000000 ) ) ;
#100865=DIRECTION ( 'NONE',  ( 0.000000000000000000, 1.000000000000000000, 0.000000000000000000 ) ) ;
#100866=CARTESIAN_POINT ( 'NONE',  ( -3.150000000000030109, 2.500000000000000000, -2.411473670974877859 ) ) ;
#100867=CARTESIAN_POINT ( 'NONE',  ( -2.300000000000033573, 12.50000000000000000, 0.2813168883297361700 ) ) ;
#100868=AXIS2_PLACEMENT_3D ( 'NONE', #102055, #63416, #12373 ) ;
#100869=AXIS2_PLACEMENT_3D ( 'NONE', #117168, #37366, #128328 ) ;
#100870=CARTESIAN_POINT ( 'NONE',  ( -3.100000000000028955, 12.50000000000000000, 4.676537180435972552 ) ) ;
#100871=VERTEX_POINT ( 'NONE', #102795 ) ;
#100872=VECTOR ( 'NONE', #32117, 1000.000000000000000 ) ;
#100873=CIRCLE ( 'NONE', #98820, 0.06509327318403745899 ) ;
#100874=ORIENTED_EDGE ( 'NONE', *, *, #29573, .T. ) ;
#100875=ORIENTED_EDGE ( 'NONE', *, *, #41140, .T. ) ;
#100876=CARTESIAN_POINT ( 'NONE',  ( -7.950000000000012612, 2.500000000000000000, 2.265063509461097357 ) ) ;
#100877=CIRCLE ( 'NONE', #17238, 0.06509327318403745899 ) ;
#100878=VERTEX_POINT ( 'NONE', #11843 ) ;
#100879=CARTESIAN_POINT ( 'NONE',  ( 17.50000000000011369, -2.362783583790017961, 3.757116699120848669 ) ) ;
#100881=AXIS2_PLACEMENT_3D ( 'NONE', #16251, #115094, #14325 ) ;
#100882=ORIENTED_EDGE ( 'NONE', *, *, #31858, .T. ) ;
#100884=DIRECTION ( 'NONE',  ( -0.000000000000000000, 1.000000000000000000, -0.000000000000000000 ) ) ;
#100885=DIRECTION ( 'NONE',  ( 0.000000000000000000, 1.000000000000000000, 0.000000000000000000 ) ) ;
#100886=CARTESIAN_POINT ( 'NONE',  ( 8.549999999999922551, 2.500000000000000000, -6.148780366869526226 ) ) ;
#100887=DIRECTION ( 'NONE',  ( 0.000000000000000000, 0.000000000000000000, 1.000000000000000000 ) ) ;
#100888=EDGE_LOOP ( 'NONE', ( #80323, #26983, #118790, #37886 ) ) ;
#100889=AXIS2_PLACEMENT_3D ( 'NONE', #80600, #21018, #100861 ) ;
#100890=CARTESIAN_POINT ( 'NONE',  ( 2.499999999999948930, 2.500000000000000000, -5.022947341949754119 ) ) ;
#100891=DIRECTION ( 'NONE',  ( 0.000000000000000000, 1.000000000000000000, 0.000000000000000000 ) ) ;
#100892=PLANE ( 'NONE',  #70135 ) ;
#100893=FACE_OUTER_BOUND ( 'NONE', #116938, .T. ) ;
#100894=ADVANCED_FACE ( 'NONE', ( #52418 ), #29107, .T. ) ;
#100896=AXIS2_PLACEMENT_3D ( 'NONE', #10752, #40922, #61180 ) ;
#100897=CONICAL_SURFACE ( 'NONE', #38237, 0.09999999999999982514, 0.003490658503988666988 ) ;
#100898=VECTOR ( 'NONE', #83164, 1000.000000000000000 ) ;
#100899=ORIENTED_EDGE ( 'NONE', *, *, #37727, .F. ) ;
#100900=DIRECTION ( 'NONE',  ( 0.000000000000000000, 0.000000000000000000, 1.000000000000000000 ) ) ;
#100901=FACE_OUTER_BOUND ( 'NONE', #10401, .T. ) ;
#100902=DIRECTION ( 'NONE',  ( -4.274815082592931898E-19, -0.9999939076577903929, -0.003490651415223739937 ) ) ;
#100904=AXIS2_PLACEMENT_3D ( 'NONE', #44504, #75255, #94899 ) ;
#100905=DIRECTION ( 'NONE',  ( -4.274815082592931898E-19, -0.9999939076577903929, -0.003490651415223739937 ) ) ;
#100906=VECTOR ( 'NONE', #128266, 1000.000000000000000 ) ;
#100907=AXIS2_PLACEMENT_3D ( 'NONE', #25199, #114867, #86040 ) ;
#100908=CARTESIAN_POINT ( 'NONE',  ( -10.20000000000000639, 2.500000000000000000, -3.983716857408421852 ) ) ;
#100909=CONICAL_SURFACE ( 'NONE', #4757, 0.1000000000000002554, 0.003490658503988666988 ) ;
#100910=EDGE_LOOP ( 'NONE', ( #70079, #47583 ) ) ;
#100911=CONICAL_SURFACE ( 'NONE', #11026, 0.1000000000000002554, 0.003490658503988666988 ) ;
#100912=AXIS2_PLACEMENT_3D ( 'NONE', #118694, #37577, #49342 ) ;
#100913=CARTESIAN_POINT ( 'NONE',  ( -11.25000000000000178, 2.500000000000000000, -1.372243186433546036 ) ) ;
#100914=ORIENTED_EDGE ( 'NONE', *, *, #25424, .F. ) ;
#100915=CIRCLE ( 'NONE', #96713, 0.06509327318403745899 ) ;
#100916=DIRECTION ( 'NONE',  ( -0.000000000000000000, -1.000000000000000000, -0.000000000000000000 ) ) ;
#100917=VERTEX_POINT ( 'NONE', #32805 ) ;
#100918=ORIENTED_EDGE ( 'NONE', *, *, #106491, .T. ) ;
#100919=FACE_OUTER_BOUND ( 'NONE', #53290, .T. ) ;
#100920=DIRECTION ( 'NONE',  ( 0.000000000000000000, -0.9999939076577903929, 0.003490651415223739937 ) ) ;
#100921=ORIENTED_EDGE ( 'NONE', *, *, #12869, .F. ) ;
#100922=ORIENTED_EDGE ( 'NONE', *, *, #8818, .F. ) ;
#100923=CARTESIAN_POINT ( 'NONE',  ( 4.599999999999940137, 12.50000000000000000, -4.330127018922201643 ) ) ;
#100924=DIRECTION ( 'NONE',  ( 0.000000000000000000, 1.000000000000000000, 0.000000000000000000 ) ) ;
#100925=EDGE_LOOP ( 'NONE', ( #91310, #30981, #28072, #109648 ) ) ;
#100926=AXIS2_PLACEMENT_3D ( 'NONE', #119404, #50679, #51354 ) ;
#100927=DIRECTION ( 'NONE',  ( 0.000000000000000000, 0.000000000000000000, -1.000000000000000000 ) ) ;
#100929=CARTESIAN_POINT ( 'NONE',  ( 10.39999999999990976, 2.500000000000000000, 4.230127018922196669 ) ) ;
#100930=DIRECTION ( 'NONE',  ( 0.000000000000000000, 0.000000000000000000, 1.000000000000000000 ) ) ;
#100931=DIRECTION ( 'NONE',  ( 0.000000000000000000, 1.000000000000000000, 0.000000000000000000 ) ) ;
#100932=DIRECTION ( 'NONE',  ( -0.000000000000000000, -1.000000000000000000, -0.000000000000000000 ) ) ;
#100933=FACE_OUTER_BOUND ( 'NONE', #58621, .T. ) ;
#100934=AXIS2_PLACEMENT_3D ( 'NONE', #64977, #15223, #35549 ) ;
#100935=AXIS2_PLACEMENT_3D ( 'NONE', #98503, #108964, #117484 ) ;
#100936=ADVANCED_FACE ( 'NONE', ( #121798 ), #6350, .T. ) ;
#100937=CIRCLE ( 'NONE', #36217, 0.06509327318403745899 ) ;
#100938=EDGE_LOOP ( 'NONE', ( #5383, #57944, #817, #41104 ) ) ;
#100940=CARTESIAN_POINT ( 'NONE',  ( -4.400000000000028777, 2.500000000000000000, -4.083716857408426826 ) ) ;
#100941=ORIENTED_EDGE ( 'NONE', *, *, #37490, .F. ) ;
#100942=CARTESIAN_POINT ( 'NONE',  ( 4.999999999999935163, 2.500000000000000000, 0.5928203230275495006 ) ) ;
#100943=DIRECTION ( 'NONE',  ( 0.000000000000000000, 1.000000000000000000, 0.000000000000000000 ) ) ;
#100944=FACE_OUTER_BOUND ( 'NONE', #104770, .T. ) ;
#100945=EDGE_LOOP ( 'NONE', ( #127235, #96148 ) ) ;
#100946=ORIENTED_EDGE ( 'NONE', *, *, #82509, .F. ) ;
#100947=EDGE_CURVE ( 'NONE', #114104, #11372, #105874, .T. ) ;
#100948=FACE_BOUND ( 'NONE', #117594, .T. ) ;
#100949=VERTEX_POINT ( 'NONE', #23604 ) ;
#100950=AXIS2_PLACEMENT_3D ( 'NONE', #67404, #65494, #66140 ) ;
#100951=EDGE_CURVE ( 'NONE', #66596, #104677, #41968, .T. ) ;
#100952=DIRECTION ( 'NONE',  ( 0.000000000000000000, 0.000000000000000000, -1.000000000000000000 ) ) ;
#100953=CARTESIAN_POINT ( 'NONE',  ( -17.50000000000000000, 1.500000000000000000, -9.999999999999998224 ) ) ;
#100954=CIRCLE ( 'NONE', #92544, 0.1000000000000002554 ) ;
#100955=CONICAL_SURFACE ( 'NONE', #65447, 0.1000000000000002554, 0.003490658503988666988 ) ;
#100956=CARTESIAN_POINT ( 'NONE',  ( 13.09999999999990195, 12.50000000000000000, -4.676537180435978769 ) ) ;
#100957=CARTESIAN_POINT ( 'NONE',  ( 16.98713617295297951, -1.503435538384354286, 5.629434171173322454 ) ) ;
#100958=AXIS2_PLACEMENT_3D ( 'NONE', #106826, #46003, #6049 ) ;
#100959=DIRECTION ( 'NONE',  ( -0.000000000000000000, -1.000000000000000000, -0.000000000000000000 ) ) ;
#100960=CARTESIAN_POINT ( 'NONE',  ( 6.899999999999928413, 2.500000000000000000, 4.676537180435972552 ) ) ;
#100961=EDGE_CURVE ( 'NONE', #96927, #129477, #33218, .T. ) ;
#100962=CARTESIAN_POINT ( 'NONE',  ( -7.500000000000001776, -2.500000000000000000, 1.734723475976807094E-15 ) ) ;
#100963=EDGE_CURVE ( 'NONE', #95314, #12469, #64582, .T. ) ;
#100964=PLANE ( 'NONE',  #35938 ) ;
#100965=EDGE_CURVE ( 'NONE', #16718, #126358, #8143, .T. ) ;
#100966=CARTESIAN_POINT ( 'NONE',  ( -0.8000000000000376810, 2.500000000000000000, -4.330127018922201643 ) ) ;
#100967=DIRECTION ( 'NONE',  ( 0.000000000000000000, -0.9999939076577903929, 0.003490651415223739937 ) ) ;
#100968=EDGE_CURVE ( 'NONE', #33066, #72150, #100102, .T. ) ;
#100969=AXIS2_PLACEMENT_3D ( 'NONE', #86254, #6386, #57467 ) ;
#100970=DIRECTION ( 'NONE',  ( 0.000000000000000000, 0.000000000000000000, 1.000000000000000000 ) ) ;
#100971=ORIENTED_EDGE ( 'NONE', *, *, #59203, .T. ) ;
#100972=VERTEX_POINT ( 'NONE', #123102 ) ;
#100973=VERTEX_POINT ( 'NONE', #26031 ) ;
#100974=AXIS2_PLACEMENT_3D ( 'NONE', #98099, #129531, #39857 ) ;
#100975=EDGE_LOOP ( 'NONE', ( #69897, #75390, #101136, #100561 ) ) ;
#100976=AXIS2_PLACEMENT_3D ( 'NONE', #33105, #92001, #112928 ) ;
#100977=AXIS2_PLACEMENT_3D ( 'NONE', #105970, #67968, #27387 ) ;
#100978=DIRECTION ( 'NONE',  ( 0.000000000000000000, 0.000000000000000000, 1.000000000000000000 ) ) ;
#100979=CARTESIAN_POINT ( 'NONE',  ( 12.49999999999993960, 2.500000000000000000, 4.330127018922196314 ) ) ;
#100980=ORIENTED_EDGE ( 'NONE', *, *, #99182, .F. ) ;
#100981=ORIENTED_EDGE ( 'NONE', *, *, #31691, .F. ) ;
#100982=ORIENTED_EDGE ( 'NONE', *, *, #35687, .F. ) ;
#100983=AXIS2_PLACEMENT_3D ( 'NONE', #71814, #11596, #80986 ) ;
#100985=DIRECTION ( 'NONE',  ( 0.000000000000000000, -0.000000000000000000, 1.000000000000000000 ) ) ;
#100986=DIRECTION ( 'NONE',  ( 0.000000000000000000, -0.000000000000000000, 1.000000000000000000 ) ) ;
#100987=DIRECTION ( 'NONE',  ( 0.000000000000000000, 0.000000000000000000, 1.000000000000000000 ) ) ;
#100988=CARTESIAN_POINT ( 'NONE',  ( -9.600000000000008527, 2.500000000000000000, 4.330127018922196314 ) ) ;
#100989=CARTESIAN_POINT ( 'NONE',  ( 9.399999999999915090, 2.500000000000000000, -4.676537180435977881 ) ) ;
#100990=CARTESIAN_POINT ( 'NONE',  ( 15.39999999999989200, 2.500000000000000000, -0.6928203230275542523 ) ) ;
#100991=ORIENTED_EDGE ( 'NONE', *, *, #9547, .T. ) ;
#100992=DIRECTION ( 'NONE',  ( 0.000000000000000000, 0.000000000000000000, 1.000000000000000000 ) ) ;
#100993=ORIENTED_EDGE ( 'NONE', *, *, #70510, .T. ) ;
#100994=ORIENTED_EDGE ( 'NONE', *, *, #4595, .T. ) ;
#100995=ORIENTED_EDGE ( 'NONE', *, *, #125327, .T. ) ;
#100996=DIRECTION ( 'NONE',  ( 0.000000000000000000, -0.000000000000000000, 1.000000000000000000 ) ) ;
#100997=VECTOR ( 'NONE', #80569, 1000.000000000000000 ) ;
#100998=CIRCLE ( 'NONE', #11096, 0.06509327318403745899 ) ;
#100999=EDGE_CURVE ( 'NONE', #14446, #45963, #60407, .T. ) ;
#101000=ORIENTED_EDGE ( 'NONE', *, *, #90362, .F. ) ;
#101001=EDGE_LOOP ( 'NONE', ( #31779, #11084, #29863, #117899 ) ) ;
#101002=EDGE_LOOP ( 'NONE', ( #108796, #17677 ) ) ;
#101003=DIRECTION ( 'NONE',  ( 0.000000000000000000, 0.000000000000000000, 1.000000000000000000 ) ) ;
#101004=DIRECTION ( 'NONE',  ( -0.000000000000000000, -1.000000000000000000, -0.000000000000000000 ) ) ;
#101006=FACE_OUTER_BOUND ( 'NONE', #120574, .T. ) ;
#101007=DIRECTION ( 'NONE',  ( 0.000000000000000000, 1.000000000000000000, 0.000000000000000000 ) ) ;
#101009=EDGE_CURVE ( 'NONE', #44822, #120717, #56268, .T. ) ;
#101010=CARTESIAN_POINT ( 'NONE',  ( -8.550000000000013145, 2.500000000000000000, 2.511473670974873507 ) ) ;
#101011=EDGE_CURVE ( 'NONE', #40034, #84934, #41635, .T. ) ;
#101012=EDGE_CURVE ( 'NONE', #103318, #58785, #114752, .T. ) ;
#101014=VERTEX_POINT ( 'NONE', #53708 ) ;
#101016=CIRCLE ( 'NONE', #117717, 0.06509327318403745899 ) ;
#101017=VERTEX_POINT ( 'NONE', #102175 ) ;
#101018=DIRECTION ( 'NONE',  ( -4.274815082592931898E-19, -0.9999939076577903929, -0.003490651415223739937 ) ) ;
#101019=LINE ( 'NONE', #121955, #18962 ) ;
#101020=CONICAL_SURFACE ( 'NONE', #29924, 0.1000000000000000472, 0.003490658503988666988 ) ;
#101021=EDGE_CURVE ( 'NONE', #12902, #10113, #129374, .T. ) ;
#101022=EDGE_LOOP ( 'NONE', ( #113640, #49967 ) ) ;
#101023=CARTESIAN_POINT ( 'NONE',  ( -13.29999999999998828, 12.50000000000000000, 4.330127018922196314 ) ) ;
#101024=EDGE_CURVE ( 'NONE', #69317, #108726, #39583, .T. ) ;
#101025=CARTESIAN_POINT ( 'NONE',  ( 15.19999999999989271, 12.50000000000000000, -0.3464101615137783474 ) ) ;
#101026=ORIENTED_EDGE ( 'NONE', *, *, #36978, .T. ) ;
#101027=AXIS2_PLACEMENT_3D ( 'NONE', #115329, #47274, #87172 ) ;
#101028=EDGE_CURVE ( 'NONE', #28470, #94678, #68795, .T. ) ;
#101029=EDGE_CURVE ( 'NONE', #51312, #47117, #16538, .T. ) ;
#101030=EDGE_CURVE ( 'NONE', #98954, #7787, #41713, .T. ) ;
#101031=CARTESIAN_POINT ( 'NONE',  ( 12.69999999999990159, 12.50000000000000000, 4.676537180435972552 ) ) ;
#101032=EDGE_LOOP ( 'NONE', ( #113143, #95904 ) ) ;
#101033=VERTEX_POINT ( 'NONE', #86868 ) ;
#101034=CARTESIAN_POINT ( 'NONE',  ( 5.849999999999934808, 2.500000000000000000, -5.802370205355749988 ) ) ;
#101035=CARTESIAN_POINT ( 'NONE',  ( 12.09999999999990195, 2.500000000000000000, 0.09999999999999772959 ) ) ;
#101036=DIRECTION ( 'NONE',  ( 0.000000000000000000, -0.9999939076577903929, 0.003490651415223739937 ) ) ;
#101037=PLANE ( 'NONE',  #11663 ) ;
#101038=EDGE_CURVE ( 'NONE', #121928, #5867, #112808, .T. ) ;
#101039=CONICAL_SURFACE ( 'NONE', #84304, 0.09999999999999982514, 0.003490658503988666988 ) ;
#101040=CARTESIAN_POINT ( 'NONE',  ( 6.699999999999928235, 2.500000000000000000, -0.1000000000000022815 ) ) ;
#101041=ORIENTED_EDGE ( 'NONE', *, *, #30551, .F. ) ;
#101042=DIRECTION ( 'NONE',  ( 0.000000000000000000, 0.000000000000000000, -1.000000000000000000 ) ) ;
#101043=CIRCLE ( 'NONE', #6923, 0.06509327318403745899 ) ;
#101044=ORIENTED_EDGE ( 'NONE', *, *, #105449, .F. ) ;
#101045=AXIS2_PLACEMENT_3D ( 'NONE', #4168, #123953, #45414 ) ;
#101046=CARTESIAN_POINT ( 'NONE',  ( 4.149999999999938183, 12.50000000000000000, 5.802370205355744659 ) ) ;
#101047=CARTESIAN_POINT ( 'NONE',  ( 10.39999999999990976, 12.50000000000000000, -4.330127018922201643 ) ) ;
#101048=AXIS2_PLACEMENT_3D ( 'NONE', #88378, #9194, #87101 ) ;
#101050=DIRECTION ( 'NONE',  ( 0.000000000000000000, 0.000000000000000000, -1.000000000000000000 ) ) ;
#101051=CARTESIAN_POINT ( 'NONE',  ( 6.249999999999965361, 2.500000000000000000, 2.165063509461097713 ) ) ;
#101052=CARTESIAN_POINT ( 'NONE',  ( 10.84999999999991260, 12.50000000000000000, 7.188010851410848723 ) ) ;
#101053=CONICAL_SURFACE ( 'NONE', #124035, 0.1000000000000000472, 0.003490658503988666988 ) ;
#101054=CARTESIAN_POINT ( 'NONE',  ( -6.250000000000021316, 2.500000000000000000, -1.372243186433550033 ) ) ;
#101055=VECTOR ( 'NONE', #101345, 1000.000000000000000 ) ;
#101056=EDGE_LOOP ( 'NONE', ( #66598, #12784 ) ) ;
#101057=CIRCLE ( 'NONE', #32215, 0.1000000000000002554 ) ;
#101058=CIRCLE ( 'NONE', #11165, 0.1000000000000002554 ) ;
#101059=CARTESIAN_POINT ( 'NONE',  ( 5.399999999999931966, 2.500000000000000000, 4.330127018922196314 ) ) ;
#101060=CARTESIAN_POINT ( 'NONE',  ( -3.950000000000024603, 12.50000000000000000, -2.511473670974877948 ) ) ;
#101061=CARTESIAN_POINT ( 'NONE',  ( -11.64999999999999680, 2.500000000000000000, -2.957883832488649833 ) ) ;
#101062=AXIS2_PLACEMENT_3D ( 'NONE', #79873, #60257, #82947 ) ;
#101063=ORIENTED_EDGE ( 'NONE', *, *, #18216, .T. ) ;
#101064=CARTESIAN_POINT ( 'NONE',  ( -3.100000000000028955, 2.500000000000000000, 3.883716857408421319 ) ) ;
#101065=ADVANCED_FACE ( 'NONE', ( #38443 ), #8236, .T. ) ;
#101066=ORIENTED_EDGE ( 'NONE', *, *, #32128, .T. ) ;
#101067=CONICAL_SURFACE ( 'NONE', #714, 0.1000000000000002554, 0.003490658503988666988 ) ;
#101068=CIRCLE ( 'NONE', #115631, 0.1000000000000000472 ) ;
#101069=ORIENTED_EDGE ( 'NONE', *, *, #16015, .F. ) ;
#101071=DIRECTION ( 'NONE',  ( 0.000000000000000000, 0.000000000000000000, -1.000000000000000000 ) ) ;
#101072=AXIS2_PLACEMENT_3D ( 'NONE', #69724, #109652, #71017 ) ;
#101073=ORIENTED_EDGE ( 'NONE', *, *, #37254, .T. ) ;
#101074=DIRECTION ( 'NONE',  ( -4.274815082592931898E-19, -0.9999939076577903929, -0.003490651415223739937 ) ) ;
#101075=LINE ( 'NONE', #80151, #38264 ) ;
#101077=EDGE_LOOP ( 'NONE', ( #62121, #21471 ) ) ;
#101078=DIRECTION ( 'NONE',  ( 0.000000000000000000, 0.000000000000000000, 1.000000000000000000 ) ) ;
#101079=DIRECTION ( 'NONE',  ( -0.000000000000000000, 1.000000000000000000, -0.000000000000000000 ) ) ;
#101080=DIRECTION ( 'NONE',  ( 0.000000000000000000, 0.000000000000000000, 1.000000000000000000 ) ) ;
#101081=EDGE_CURVE ( 'NONE', #22839, #111368, #87653, .T. ) ;
#101082=ORIENTED_EDGE ( 'NONE', *, *, #89326, .T. ) ;
#101083=EDGE_LOOP ( 'NONE', ( #57800, #34646, #74383, #54252 ) ) ;
#101084=ORIENTED_EDGE ( 'NONE', *, *, #102730, .T. ) ;
#101085=CARTESIAN_POINT ( 'NONE',  ( -0.6500000000000389910, 2.500000000000000000, -1.818653347947326138 ) ) ;
#101086=PLANE ( 'NONE',  #54185 ) ;
#101087=CIRCLE ( 'NONE', #73896, 0.1000000000000002554 ) ;
#101088=DIRECTION ( 'NONE',  ( 0.000000000000000000, 0.000000000000000000, -1.000000000000000000 ) ) ;
#101089=AXIS2_PLACEMENT_3D ( 'NONE', #34662, #65373, #33997 ) ;
#101090=FACE_BOUND ( 'NONE', #68742, .T. ) ;
#101091=ORIENTED_EDGE ( 'NONE', *, *, #15659, .T. ) ;
#101092=DIRECTION ( 'NONE',  ( 0.000000000000000000, 1.000000000000000000, 0.000000000000000000 ) ) ;
#101093=CARTESIAN_POINT ( 'NONE',  ( -0.8500000000000382805, 2.500000000000000000, -5.902370205355750521 ) ) ;
#101094=ORIENTED_EDGE ( 'NONE', *, *, #129344, .T. ) ;
#101095=CARTESIAN_POINT ( 'NONE',  ( -0.8500000000000395017, 12.50000000000000000, 6.495190528383297135 ) ) ;
#101096=CARTESIAN_POINT ( 'NONE',  ( 17.49149641758760509, 2.499999999999969358, 4.292093396892645352 ) ) ;
#101097=AXIS2_PLACEMENT_3D ( 'NONE', #33896, #75113, #105206 ) ;
#101098=AXIS2_PLACEMENT_3D ( 'NONE', #101316, #11634, #43703 ) ;
#101099=DIRECTION ( 'NONE',  ( 0.000000000000000000, 0.000000000000000000, 1.000000000000000000 ) ) ;
#101100=AXIS2_PLACEMENT_3D ( 'NONE', #103618, #15858, #115998 ) ;
#101101=DIRECTION ( 'NONE',  ( 0.000000000000000000, 1.000000000000000000, 0.000000000000000000 ) ) ;
#101102=DIRECTION ( 'NONE',  ( 0.000000000000000000, 0.000000000000000000, -1.000000000000000000 ) ) ;
#101103=CARTESIAN_POINT ( 'NONE',  ( -8.300000000000011369, 2.500000000000000000, -2.276824562219559311E-15 ) ) ;
#101104=CARTESIAN_POINT ( 'NONE',  ( 2.299999999999948752, 2.500000000000000000, -3.983716857408426293 ) ) ;
#101105=VECTOR ( 'NONE', #11851, 1000.000000000000000 ) ;
#101106=AXIS2_PLACEMENT_3D ( 'NONE', #109527, #1490, #51902 ) ;
#101107=AXIS2_PLACEMENT_3D ( 'NONE', #85318, #35590, #66319 ) ;
#101108=EDGE_CURVE ( 'NONE', #126341, #83526, #33310, .T. ) ;
#101109=ORIENTED_EDGE ( 'NONE', *, *, #73504, .T. ) ;
#101110=ORIENTED_EDGE ( 'NONE', *, *, #22512, .F. ) ;
#101111=ORIENTED_EDGE ( 'NONE', *, *, #49281, .T. ) ;
#101113=DIRECTION ( 'NONE',  ( 0.000000000000000000, 1.000000000000000000, 0.000000000000000000 ) ) ;
#101114=VECTOR ( 'NONE', #70, 1000.000000000000000 ) ;
#101115=CARTESIAN_POINT ( 'NONE',  ( -8.749999999999976907, 12.50000000000000000, -6.560283801567334372 ) ) ;
#101116=EDGE_LOOP ( 'NONE', ( #108939, #30817 ) ) ;
#101117=FACE_BOUND ( 'NONE', #52006, .T. ) ;
#101118=ADVANCED_FACE ( 'NONE', ( #67870 ), #121116, .T. ) ;
#101119=DIRECTION ( 'NONE',  ( -0.000000000000000000, 1.000000000000000000, -0.000000000000000000 ) ) ;
#101120=DIRECTION ( 'NONE',  ( -4.274815082592931898E-19, -0.9999939076577903929, -0.003490651415223739937 ) ) ;
#101121=LINE ( 'NONE', #7074, #111858 ) ;
#101122=DIRECTION ( 'NONE',  ( 0.000000000000000000, 0.000000000000000000, -1.000000000000000000 ) ) ;
#101123=DIRECTION ( 'NONE',  ( -0.000000000000000000, -1.000000000000000000, -0.000000000000000000 ) ) ;
#101124=EDGE_CURVE ( 'NONE', #124699, #120570, #31245, .T. ) ;
#101125=CARTESIAN_POINT ( 'NONE',  ( 12.69999999999989981, 12.50000000000000000, -0.3464101615137783474 ) ) ;
#101126=ADVANCED_FACE ( 'NONE', ( #118262 ), #127385, .T. ) ;
#101127=PLANE ( 'NONE',  #104006 ) ;
#101128=CARTESIAN_POINT ( 'NONE',  ( -1.850000000000033396, 12.50000000000000000, -1.818653347947325916 ) ) ;
#101129=EDGE_CURVE ( 'NONE', #51103, #16412, #62638, .T. ) ;
#101130=CARTESIAN_POINT ( 'NONE',  ( 12.49999999999990408, 12.50000000000000000, -3.637306695894650055 ) ) ;
#101131=EDGE_CURVE ( 'NONE', #59733, #88940, #79363, .T. ) ;
#101132=ORIENTED_EDGE ( 'NONE', *, *, #1122, .T. ) ;
#101133=ADVANCED_FACE ( 'NONE', ( #79011 ), #22927, .T. ) ;
#101134=CIRCLE ( 'NONE', #63477, 0.1000000000000000056 ) ;
#101135=ORIENTED_EDGE ( 'NONE', *, *, #90865, .F. ) ;
#101136=ORIENTED_EDGE ( 'NONE', *, *, #46305, .T. ) ;
#101137=ORIENTED_EDGE ( 'NONE', *, *, #57677, .F. ) ;
#101138=VERTEX_POINT ( 'NONE', #67194 ) ;
#101139=ORIENTED_EDGE ( 'NONE', *, *, #25077, .T. ) ;
#101140=DIRECTION ( 'NONE',  ( 0.000000000000000000, 0.000000000000000000, 1.000000000000000000 ) ) ;
#101141=ORIENTED_EDGE ( 'NONE', *, *, #105582, .T. ) ;
#101142=EDGE_CURVE ( 'NONE', #126312, #103698, #18124, .T. ) ;
#101143=VECTOR ( 'NONE', #91400, 1000.000000000000000 ) ;
#101144=CIRCLE ( 'NONE', #44714, 0.1000000000000002554 ) ;
#101145=EDGE_CURVE ( 'NONE', #113182, #72573, #87501, .T. ) ;
#101146=VECTOR ( 'NONE', #78236, 1000.000000000000000 ) ;
#101147=ADVANCED_FACE ( 'NONE', ( #88130 ), #58436, .T. ) ;
#101148=CARTESIAN_POINT ( 'NONE',  ( 16.86635082839116606, 0.4716143926291154198, 5.778906370536208925 ) ) ;
#101149=CARTESIAN_POINT ( 'NONE',  ( 13.51931942407985332, -1.499999999999904521, 8.074217333073772096 ) ) ;
#101150=DIRECTION ( 'NONE',  ( 0.000000000000000000, -0.9999939076577903929, 0.003490651415223739937 ) ) ;
#101151=CARTESIAN_POINT ( 'NONE',  ( -3.550000000000031797, 12.50000000000000000, -6.083687093685488989 ) ) ;
#101152=CIRCLE ( 'NONE', #34266, 0.09999999999999999167 ) ;
#101153=ORIENTED_EDGE ( 'NONE', *, *, #82726, .F. ) ;
#101154=CARTESIAN_POINT ( 'NONE',  ( 1.649999999999951505, 12.50000000000000000, -2.922977105672691422 ) ) ;
#101155=CIRCLE ( 'NONE', #42588, 0.1000000000000002554 ) ;
#101156=VECTOR ( 'NONE', #74913, 1000.000000000000000 ) ;
#101157=ORIENTED_EDGE ( 'NONE', *, *, #15949, .F. ) ;
#101158=CIRCLE ( 'NONE', #101239, 0.1000000000000002554 ) ;
#101159=ORIENTED_EDGE ( 'NONE', *, *, #67985, .T. ) ;
#101160=LINE ( 'NONE', #51430, #34313 ) ;
#101161=DIRECTION ( 'NONE',  ( 0.000000000000000000, 0.000000000000000000, 1.000000000000000000 ) ) ;
#101162=CARTESIAN_POINT ( 'NONE',  ( 8.549999999999918998, 2.500000000000000000, 6.841600689897072485 ) ) ;
#101163=AXIS2_PLACEMENT_3D ( 'NONE', #127380, #114956, #96600 ) ;
#101164=ORIENTED_EDGE ( 'NONE', *, *, #2482, .F. ) ;
#101165=VERTEX_POINT ( 'NONE', #37780 ) ;
#101166=DIRECTION ( 'NONE',  ( 0.000000000000000000, 0.000000000000000000, 1.000000000000000000 ) ) ;
#101167=DIRECTION ( 'NONE',  ( 0.000000000000000000, 1.000000000000000000, 0.000000000000000000 ) ) ;
#101168=CARTESIAN_POINT ( 'NONE',  ( -10.65000000000000213, 12.50000000000000000, 2.511473670974873507 ) ) ;
#101169=DIRECTION ( 'NONE',  ( -0.000000000000000000, 1.000000000000000000, -0.000000000000000000 ) ) ;
#101170=VERTEX_POINT ( 'NONE', #98603 ) ;
#101171=DIRECTION ( 'NONE',  ( 0.000000000000000000, 1.000000000000000000, 0.000000000000000000 ) ) ;
#101172=AXIS2_PLACEMENT_3D ( 'NONE', #42201, #978, #93235 ) ;
#101173=ORIENTED_EDGE ( 'NONE', *, *, #75766, .F. ) ;
#101174=CONICAL_SURFACE ( 'NONE', #42705, 0.1000000000000002554, 0.003490658503988666988 ) ;
#101175=FACE_OUTER_BOUND ( 'NONE', #45260, .T. ) ;
#101176=ORIENTED_EDGE ( 'NONE', *, *, #113779, .T. ) ;
#101178=CARTESIAN_POINT ( 'NONE',  ( 1.849999999999949019, 2.500000000000000000, 6.841600689897072485 ) ) ;
#101179=CARTESIAN_POINT ( 'NONE',  ( 3.549999999999943867, 2.500000000000000000, -6.148780366869526226 ) ) ;
#101180=EDGE_CURVE ( 'NONE', #40494, #108185, #77208, .T. ) ;
#101181=DIRECTION ( 'NONE',  ( 0.000000000000000000, 1.000000000000000000, 0.000000000000000000 ) ) ;
#101182=VERTEX_POINT ( 'NONE', #78362 ) ;
#101183=ADVANCED_FACE ( 'NONE', ( #8942 ), #75149, .T. ) ;
#101184=CARTESIAN_POINT ( 'NONE',  ( -5.850000000000019185, 2.500000000000000000, 2.065063509461097624 ) ) ;
#101186=CARTESIAN_POINT ( 'NONE',  ( 9.999999999999948486, 2.500000000000000000, 4.430127018922196847 ) ) ;
#101187=EDGE_LOOP ( 'NONE', ( #93267, #7627 ) ) ;
#101188=ORIENTED_EDGE ( 'NONE', *, *, #74344, .F. ) ;
#101189=CONICAL_SURFACE ( 'NONE', #13335, 0.1000000000000000056, 0.003490658503988666988 ) ;
#101190=VECTOR ( 'NONE', #128182, 1000.000000000000000 ) ;
#101191=ORIENTED_EDGE ( 'NONE', *, *, #2026, .T. ) ;
#101192=CARTESIAN_POINT ( 'NONE',  ( 17.50000000000000000, -0.9166666666666694052, 4.000000000000001776 ) ) ;
#101193=CARTESIAN_POINT ( 'NONE',  ( 1.899999999999951283, 2.500000000000000000, -4.676537180435977881 ) ) ;
#101194=CARTESIAN_POINT ( 'NONE',  ( 20.59313469514023964, 2.666874593322334341, 2.243770147468749698 ) ) ;
#101195=DIRECTION ( 'NONE',  ( -0.000000000000000000, 1.000000000000000000, -0.000000000000000000 ) ) ;
#101196=CARTESIAN_POINT ( 'NONE',  ( 2.299999999999947864, 2.500000000000000000, 3.883716857408421319 ) ) ;
#101197=EDGE_CURVE ( 'NONE', #48618, #56136, #127453, .T. ) ;
#101198=CARTESIAN_POINT ( 'NONE',  ( -8.300000000000011369, 2.500000000000000000, -4.330127018922201643 ) ) ;
#101199=CIRCLE ( 'NONE', #9253, 0.09999999999999982514 ) ;
#101200=DIRECTION ( 'NONE',  ( 0.000000000000000000, 0.000000000000000000, 1.000000000000000000 ) ) ;
#101201=AXIS2_PLACEMENT_3D ( 'NONE', #29734, #27153, #67050 ) ;
#101202=DIRECTION ( 'NONE',  ( 0.000000000000000000, 0.000000000000000000, 1.000000000000000000 ) ) ;
#101203=DIRECTION ( 'NONE',  ( 0.000000000000000000, 0.000000000000000000, -1.000000000000000000 ) ) ;
#101204=VECTOR ( 'NONE', #98252, 1000.000000000000000 ) ;
#101205=AXIS2_PLACEMENT_3D ( 'NONE', #122325, #112497, #20889 ) ;
#101206=VECTOR ( 'NONE', #12594, 1000.000000000000000 ) ;
#101207=CIRCLE ( 'NONE', #92903, 0.09999999999999999167 ) ;
#101208=EDGE_LOOP ( 'NONE', ( #66685, #47876, #129188, #40329 ) ) ;
#101210=CARTESIAN_POINT ( 'NONE',  ( -1.850000000000033396, 2.500000000000000000, -6.048780366869526581 ) ) ;
#101211=EDGE_CURVE ( 'NONE', #13926, #48067, #123180, .T. ) ;
#101212=CARTESIAN_POINT ( 'NONE',  ( -1.250000000000037526, 12.50000000000000000, -5.737276932171712751 ) ) ;
#101213=DIRECTION ( 'NONE',  ( 0.000000000000000000, 1.000000000000000000, 0.000000000000000000 ) ) ;
#101215=FACE_OUTER_BOUND ( 'NONE', #43716, .T. ) ;
#101216=DIRECTION ( 'NONE',  ( 0.000000000000000000, 0.000000000000000000, 1.000000000000000000 ) ) ;
#101217=LINE ( 'NONE', #41028, #104788 ) ;
#101218=ORIENTED_EDGE ( 'NONE', *, *, #3767, .T. ) ;
#101219=AXIS2_PLACEMENT_3D ( 'NONE', #33558, #3433, #82656 ) ;
#101220=VECTOR ( 'NONE', #38648, 1000.000000000000000 ) ;
#101221=VERTEX_POINT ( 'NONE', #50195 ) ;
#101223=ADVANCED_FACE ( 'NONE', ( #71754 ), #52163, .T. ) ;
#101224=ORIENTED_EDGE ( 'NONE', *, *, #80353, .F. ) ;
#101225=VERTEX_POINT ( 'NONE', #79632 ) ;
#101226=DIRECTION ( 'NONE',  ( -0.000000000000000000, 1.000000000000000000, -0.000000000000000000 ) ) ;
#101227=FACE_OUTER_BOUND ( 'NONE', #121411, .T. ) ;
#101228=CARTESIAN_POINT ( 'NONE',  ( 2.299999999999949640, 2.500000000000000000, -0.3464101615137782364 ) ) ;
#101229=VECTOR ( 'NONE', #44280, 1000.000000000000000 ) ;
#101230=CARTESIAN_POINT ( 'NONE',  ( 14.39999999999989555, 2.500000000000000000, 0.2464101615137736789 ) ) ;
#101231=AXIS2_PLACEMENT_3D ( 'NONE', #47162, #97534, #5282 ) ;
#101232=ORIENTED_EDGE ( 'NONE', *, *, #16495, .F. ) ;
#101233=DIRECTION ( 'NONE',  ( 0.000000000000000000, 1.000000000000000000, 0.000000000000000000 ) ) ;
#101234=EDGE_LOOP ( 'NONE', ( #116643, #62531 ) ) ;
#101235=CARTESIAN_POINT ( 'NONE',  ( 16.96615051717511591, 1.026750547576220862, 5.590381354649148093 ) ) ;
#101236=ADVANCED_FACE ( 'NONE', ( #60020 ), #60654, .T. ) ;
#101237=CARTESIAN_POINT ( 'NONE',  ( 3.149999999999942624, 2.500000000000000000, 6.741600689897071952 ) ) ;
#101238=EDGE_LOOP ( 'NONE', ( #502, #127855, #61160, #36117 ) ) ;
#101239=AXIS2_PLACEMENT_3D ( 'NONE', #98463, #117442, #97832 ) ;
#101240=ORIENTED_EDGE ( 'NONE', *, *, #113883, .T. ) ;
#101241=ORIENTED_EDGE ( 'NONE', *, *, #93511, .T. ) ;
#101242=ORIENTED_EDGE ( 'NONE', *, *, #53819, .F. ) ;
#101243=DIRECTION ( 'NONE',  ( 0.000000000000000000, 1.000000000000000000, 0.000000000000000000 ) ) ;
#101244=CARTESIAN_POINT ( 'NONE',  ( 8.340322510126762623, 2.500000000000001332, 8.517653997967753909 ) ) ;
#101245=CARTESIAN_POINT ( 'NONE',  ( 3.099999999999945022, 2.500000000000000000, -0.3464101615137783474 ) ) ;
#101246=FACE_BOUND ( 'NONE', #24698, .T. ) ;
#101247=FACE_OUTER_BOUND ( 'NONE', #70465, .T. ) ;
#101249=CARTESIAN_POINT ( 'NONE',  ( 11.24999999999990941, 2.500000000000000000, 7.188010851410848723 ) ) ;
#101250=CARTESIAN_POINT ( 'NONE',  ( -8.350000000000013856, 12.50000000000000000, -5.802370205355744659 ) ) ;
#101251=AXIS2_PLACEMENT_3D ( 'NONE', #110730, #2061, #111363 ) ;
#101252=CIRCLE ( 'NONE', #99208, 0.1000000000000002554 ) ;
#101253=DIRECTION ( 'NONE',  ( 0.000000000000000000, 0.000000000000000000, 1.000000000000000000 ) ) ;
#101254=CARTESIAN_POINT ( 'NONE',  ( -13.14999999999999147, 2.500000000000000000, -2.611473670974875372 ) ) ;
#101255=AXIS2_PLACEMENT_3D ( 'NONE', #93715, #23685, #63620 ) ;
#101256=DIRECTION ( 'NONE',  ( 0.000000000000000000, 0.000000000000000000, 1.000000000000000000 ) ) ;
#101257=VECTOR ( 'NONE', #73079, 1000.000000000000000 ) ;
#101258=CARTESIAN_POINT ( 'NONE',  ( -5.850000000000021849, 12.50000000000000000, -1.472243186433550122 ) ) ;
#101259=ADVANCED_FACE ( 'NONE', ( #20077 ), #29199, .T. ) ;
#101260=VERTEX_POINT ( 'NONE', #2337 ) ;
#101261=ORIENTED_EDGE ( 'NONE', *, *, #40395, .F. ) ;
#101262=VERTEX_POINT ( 'NONE', #40371 ) ;
#101263=ORIENTED_EDGE ( 'NONE', *, *, #83606, .F. ) ;
#101264=EDGE_LOOP ( 'NONE', ( #119926, #10785 ) ) ;
#101265=DIRECTION ( 'NONE',  ( -0.000000000000000000, 1.000000000000000000, -0.000000000000000000 ) ) ;
#101266=DIRECTION ( 'NONE',  ( 0.000000000000000000, 1.000000000000000000, 0.000000000000000000 ) ) ;
#101267=ORIENTED_EDGE ( 'NONE', *, *, #31527, .F. ) ;
#101268=FACE_BOUND ( 'NONE', #98038, .T. ) ;
#101269=FACE_OUTER_BOUND ( 'NONE', #25117, .T. ) ;
#101270=EDGE_CURVE ( 'NONE', #125301, #76186, #45908, .T. ) ;
#101271=AXIS2_PLACEMENT_3D ( 'NONE', #32140, #101509, #89107 ) ;
#101272=AXIS2_PLACEMENT_3D ( 'NONE', #83010, #41806, #84274 ) ;
#101274=ORIENTED_EDGE ( 'NONE', *, *, #52932, .F. ) ;
#101275=EDGE_CURVE ( 'NONE', #57444, #48343, #80289, .T. ) ;
#101276=DIRECTION ( 'NONE',  ( 0.000000000000000000, 0.000000000000000000, 1.000000000000000000 ) ) ;
#101277=VECTOR ( 'NONE', #27370, 1000.000000000000000 ) ;
#101278=CARTESIAN_POINT ( 'NONE',  ( 5.199999999999937117, 12.50000000000000000, -4.741630453620016006 ) ) ;
#101279=EDGE_CURVE ( 'NONE', #29350, #102543, #119065, .T. ) ;
#101280=CARTESIAN_POINT ( 'NONE',  ( -2.050000000000032685, 2.500000000000000000, -2.165063509461101710 ) ) ;
#101281=EDGE_CURVE ( 'NONE', #97971, #115638, #96069, .T. ) ;
#101282=DIRECTION ( 'NONE',  ( 0.000000000000000000, 0.000000000000000000, -1.000000000000000000 ) ) ;
#101283=EDGE_CURVE ( 'NONE', #39915, #103444, #39670, .T. ) ;
#101284=ORIENTED_EDGE ( 'NONE', *, *, #123031, .T. ) ;
#101285=CARTESIAN_POINT ( 'NONE',  ( 4.149999999999939959, 2.500000000000000000, -2.265063509461101798 ) ) ;
#101286=CONICAL_SURFACE ( 'NONE', #124275, 0.09999999999999999167, 0.003490658503988666988 ) ;
#101287=CIRCLE ( 'NONE', #28132, 0.06509327318403745899 ) ;
#101289=ORIENTED_EDGE ( 'NONE', *, *, #25069, .T. ) ;
#101290=EDGE_CURVE ( 'NONE', #6486, #34419, #70943, .T. ) ;
#101291=ORIENTED_EDGE ( 'NONE', *, *, #109246, .T. ) ;
#101292=LINE ( 'NONE', #21430, #80063 ) ;
#101293=EDGE_CURVE ( 'NONE', #95559, #99317, #43774, .T. ) ;
#101294=CARTESIAN_POINT ( 'NONE',  ( 3.349999999999945466, 12.50000000000000000, -2.165063509461101710 ) ) ;
#101295=ORIENTED_EDGE ( 'NONE', *, *, #63331, .F. ) ;
#101296=ADVANCED_FACE ( 'NONE', ( #99928 ), #102498, .T. ) ;
#101297=CARTESIAN_POINT ( 'NONE',  ( -12.09999999999999609, 2.500000000000000000, -4.330127018922198978 ) ) ;
#101298=ADVANCED_FACE ( 'NONE', ( #90080 ), #110377, .T. ) ;
#101299=AXIS2_PLACEMENT_3D ( 'NONE', #52249, #122285, #40514 ) ;
#101300=AXIS2_PLACEMENT_3D ( 'NONE', #31415, #1293, #41244 ) ;
#101301=CARTESIAN_POINT ( 'NONE',  ( -4.999999999999986677, 12.50000000000000000, -2.276824562219559311E-15 ) ) ;
#101302=ADVANCED_FACE ( 'NONE', ( #10859 ), #89453, .T. ) ;
#101303=CARTESIAN_POINT ( 'NONE',  ( -4.350000000000023626, 12.50000000000000000, 2.576566944158910744 ) ) ;
#101304=CARTESIAN_POINT ( 'NONE',  ( 6.649999999999931966, 2.500000000000000000, -5.702370205355749455 ) ) ;
#101306=AXIS2_PLACEMENT_3D ( 'NONE', #59361, #68504, #1692 ) ;
#101307=ORIENTED_EDGE ( 'NONE', *, *, #3861, .F. ) ;
#101308=DIRECTION ( 'NONE',  ( 0.000000000000000000, 0.000000000000000000, 1.000000000000000000 ) ) ;
#101309=EDGE_CURVE ( 'NONE', #103801, #126753, #94013, .T. ) ;
#101310=ORIENTED_EDGE ( 'NONE', *, *, #66656, .F. ) ;
#101311=FACE_OUTER_BOUND ( 'NONE', #73782, .T. ) ;
#101312=ORIENTED_EDGE ( 'NONE', *, *, #2526, .T. ) ;
#101313=CARTESIAN_POINT ( 'NONE',  ( 5.599999999999934808, 2.500000000000000000, -4.576537180435978236 ) ) ;
#101314=EDGE_LOOP ( 'NONE', ( #86061, #8403 ) ) ;
#101315=LINE ( 'NONE', #90839, #9510 ) ;
#101316=CARTESIAN_POINT ( 'NONE',  ( 7.099999999999926814, 2.500000000000000000, -2.276824562219559311E-15 ) ) ;
#101317=DIRECTION ( 'NONE',  ( -0.000000000000000000, -1.000000000000000000, -0.000000000000000000 ) ) ;
#101318=DIRECTION ( 'NONE',  ( 0.000000000000000000, -0.9999939076577903929, 0.003490651415223739937 ) ) ;
#101319=DIRECTION ( 'NONE',  ( -0.000000000000000000, -1.000000000000000000, -0.000000000000000000 ) ) ;
#101320=AXIS2_PLACEMENT_3D ( 'NONE', #83334, #73483, #45342 ) ;
#101321=VERTEX_POINT ( 'NONE', #11532 ) ;
#101322=EDGE_LOOP ( 'NONE', ( #94692, #119295, #115509, #103375 ) ) ;
#101323=ORIENTED_EDGE ( 'NONE', *, *, #69206, .T. ) ;
#101324=DIRECTION ( 'NONE',  ( -0.000000000000000000, 1.000000000000000000, -0.000000000000000000 ) ) ;
#101325=DIRECTION ( 'NONE',  ( 0.000000000000000000, 0.000000000000000000, 1.000000000000000000 ) ) ;
#101326=DIRECTION ( 'NONE',  ( 0.000000000000000000, 0.000000000000000000, 1.000000000000000000 ) ) ;
#101327=ORIENTED_EDGE ( 'NONE', *, *, #49119, .T. ) ;
#101328=ORIENTED_EDGE ( 'NONE', *, *, #19974, .T. ) ;
#101329=EDGE_LOOP ( 'NONE', ( #104948, #64114, #100995, #110289 ) ) ;
#101330=CARTESIAN_POINT ( 'NONE',  ( 6.249999999999932498, 2.500000000000000000, -5.702370205355749455 ) ) ;
#101331=CONICAL_SURFACE ( 'NONE', #63681, 0.1000000000000002554, 0.003490658503988666988 ) ;
#101332=ORIENTED_EDGE ( 'NONE', *, *, #16609, .F. ) ;
#101333=DIRECTION ( 'NONE',  ( 0.000000000000000000, 1.000000000000000000, 0.000000000000000000 ) ) ;
#101334=DIRECTION ( 'NONE',  ( -0.000000000000000000, -1.000000000000000000, -0.000000000000000000 ) ) ;
#101335=AXIS2_PLACEMENT_3D ( 'NONE', #13661, #94165, #32050 ) ;
#101336=CARTESIAN_POINT ( 'NONE',  ( -10.85000000000000142, 2.500000000000000000, -7.288010851410851032 ) ) ;
#101337=DIRECTION ( 'NONE',  ( 0.000000000000000000, 0.000000000000000000, -1.000000000000000000 ) ) ;
#101338=CARTESIAN_POINT ( 'NONE',  ( 10.39999999999991331, 2.500000000000000000, -0.1000000000000023925 ) ) ;
#101339=CARTESIAN_POINT ( 'NONE',  ( 11.04999999999990834, 2.500000000000000000, -6.941600689897077459 ) ) ;
#101340=DIRECTION ( 'NONE',  ( 0.000000000000000000, 0.000000000000000000, 1.000000000000000000 ) ) ;
#101341=FACE_OUTER_BOUND ( 'NONE', #69627, .T. ) ;
#101342=ORIENTED_EDGE ( 'NONE', *, *, #91388, .F. ) ;
#101343=AXIS2_PLACEMENT_3D ( 'NONE', #113459, #62446, #44735 ) ;
#101344=EDGE_CURVE ( 'NONE', #117711, #27277, #51474, .T. ) ;
#101345=DIRECTION ( 'NONE',  ( 0.000000000000000000, -0.9999939076577903929, 0.003490651415223739937 ) ) ;
#101346=DIRECTION ( 'NONE',  ( 0.000000000000000000, 0.000000000000000000, 1.000000000000000000 ) ) ;
#101347=CONICAL_SURFACE ( 'NONE', #113861, 0.09999999999999999167, 0.003490658503988666988 ) ;
#101348=EDGE_CURVE ( 'NONE', #40443, #83814, #112322, .T. ) ;
#101349=EDGE_LOOP ( 'NONE', ( #102579, #8014 ) ) ;
#101350=VERTEX_POINT ( 'NONE', #124064 ) ;
#101352=LINE ( 'NONE', #30039, #48987 ) ;
#101353=DIRECTION ( 'NONE',  ( 0.000000000000000000, 0.000000000000000000, 1.000000000000000000 ) ) ;
#101354=DIRECTION ( 'NONE',  ( 0.000000000000000000, 1.000000000000000000, 0.000000000000000000 ) ) ;
#101355=EDGE_CURVE ( 'NONE', #46558, #92955, #8327, .T. ) ;
#101356=DIRECTION ( 'NONE',  ( 0.000000000000000000, 1.000000000000000000, 0.000000000000000000 ) ) ;
#101357=CONICAL_SURFACE ( 'NONE', #82578, 0.09999999999999982514, 0.003490658503988666988 ) ;
#101358=PLANE ( 'NONE',  #42815 ) ;
#101359=AXIS2_PLACEMENT_3D ( 'NONE', #2257, #3563, #13377 ) ;
#101360=CARTESIAN_POINT ( 'NONE',  ( -2.700000000000031264, 12.50000000000000000, 4.676537180435972552 ) ) ;
#101361=DIRECTION ( 'NONE',  ( 0.000000000000000000, -0.000000000000000000, 1.000000000000000000 ) ) ;
#101362=CIRCLE ( 'NONE', #57439, 0.1000000000000002554 ) ;
#101363=CIRCLE ( 'NONE', #97149, 0.1000000000000002554 ) ;
#101364=FACE_OUTER_BOUND ( 'NONE', #17247, .T. ) ;
#101365=EDGE_LOOP ( 'NONE', ( #44156, #59316 ) ) ;
#101366=VERTEX_POINT ( 'NONE', #23280 ) ;
#101367=EDGE_LOOP ( 'NONE', ( #23338, #24804, #125501, #21601 ) ) ;
#101368=ORIENTED_EDGE ( 'NONE', *, *, #83322, .T. ) ;
#101369=DIRECTION ( 'NONE',  ( 0.000000000000000000, -0.000000000000000000, 1.000000000000000000 ) ) ;
#101370=CARTESIAN_POINT ( 'NONE',  ( -7.700000000000014388, 2.500000000000000000, -4.676537180435977881 ) ) ;
#101371=ORIENTED_EDGE ( 'NONE', *, *, #73505, .F. ) ;
#101372=PLANE ( 'NONE',  #128022 ) ;
#101373=DIRECTION ( 'NONE',  ( 0.000000000000000000, 0.000000000000000000, -1.000000000000000000 ) ) ;
#101374=CIRCLE ( 'NONE', #44937, 0.1000000000000002554 ) ;
#101375=DIRECTION ( 'NONE',  ( 0.000000000000000000, 1.000000000000000000, 0.000000000000000000 ) ) ;
#101376=FACE_OUTER_BOUND ( 'NONE', #3291, .T. ) ;
#101377=ORIENTED_EDGE ( 'NONE', *, *, #68482, .F. ) ;
#101378=CONICAL_SURFACE ( 'NONE', #13526, 0.09999999999999982514, 0.003490658503988666988 ) ;
#101379=FACE_OUTER_BOUND ( 'NONE', #81713, .T. ) ;
#101380=CARTESIAN_POINT ( 'NONE',  ( -1.650000000000034328, 2.500000000000000000, -2.165063509461101710 ) ) ;
#101381=EDGE_CURVE ( 'NONE', #71296, #18587, #60593, .T. ) ;
#101382=ORIENTED_EDGE ( 'NONE', *, *, #14651, .T. ) ;
#101384=CIRCLE ( 'NONE', #88855, 0.06509327318403745899 ) ;
#101385=AXIS2_PLACEMENT_3D ( 'NONE', #71550, #121948, #23102 ) ;
#101386=ORIENTED_EDGE ( 'NONE', *, *, #97458, .F. ) ;
#101387=ORIENTED_EDGE ( 'NONE', *, *, #82218, .T. ) ;
#101388=VERTEX_POINT ( 'NONE', #122782 ) ;
#101389=CARTESIAN_POINT ( 'NONE',  ( -10.45000000000000462, 12.50000000000000000, -6.495190528383298911 ) ) ;
#101390=DIRECTION ( 'NONE',  ( -0.000000000000000000, 1.000000000000000000, -0.000000000000000000 ) ) ;
#101391=CARTESIAN_POINT ( 'NONE',  ( 2.500000000000001332, -2.392226903609812716, -9.521986658763280431 ) ) ;
#101392=CIRCLE ( 'NONE', #38723, 0.1000000000000002554 ) ;
#101393=CIRCLE ( 'NONE', #70091, 0.09999999999999982514 ) ;
#101394=ORIENTED_EDGE ( 'NONE', *, *, #43661, .T. ) ;
#101395=CARTESIAN_POINT ( 'NONE',  ( 2.899999999999944844, 2.500000000000000000, 5.022947341949748790 ) ) ;
#101396=AXIS2_PLACEMENT_3D ( 'NONE', #15859, #116000, #95731 ) ;
#101397=EDGE_CURVE ( 'NONE', #46092, #72427, #54312, .T. ) ;
#101398=ORIENTED_EDGE ( 'NONE', *, *, #36160, .F. ) ;
#101399=DIRECTION ( 'NONE',  ( 0.000000000000000000, 1.000000000000000000, 0.000000000000000000 ) ) ;
#101400=CARTESIAN_POINT ( 'NONE',  ( 17.19804440726981198, -0.4677972980984271834, -5.492654682185318826 ) ) ;
#101401=DIRECTION ( 'NONE',  ( 0.000000000000000000, 0.000000000000000000, 1.000000000000000000 ) ) ;
#101402=DIRECTION ( 'NONE',  ( 0.000000000000000000, 0.000000000000000000, -1.000000000000000000 ) ) ;
#101403=EDGE_CURVE ( 'NONE', #97815, #24862, #66806, .T. ) ;
#101404=ORIENTED_EDGE ( 'NONE', *, *, #57059, .T. ) ;
#101405=ORIENTED_EDGE ( 'NONE', *, *, #46855, .F. ) ;
#101406=VERTEX_POINT ( 'NONE', #65783 ) ;
#101407=DIRECTION ( 'NONE',  ( 0.000000000000000000, 0.000000000000000000, 1.000000000000000000 ) ) ;
#101408=EDGE_CURVE ( 'NONE', #101653, #62839, #98210, .T. ) ;
#101409=DIRECTION ( 'NONE',  ( 0.000000000000000000, 0.000000000000000000, 1.000000000000000000 ) ) ;
#101410=FACE_BOUND ( 'NONE', #160, .T. ) ;
#101411=CARTESIAN_POINT ( 'NONE',  ( 12.09999999999990550, 12.50000000000000000, -3.702399969078687292 ) ) ;
#101412=AXIS2_PLACEMENT_3D ( 'NONE', #99026, #89201, #11279 ) ;
#101413=CARTESIAN_POINT ( 'NONE',  ( 0.8499999999999553468, 12.50000000000000000, -2.857883832488653741 ) ) ;
#101414=DIRECTION ( 'NONE',  ( 0.000000000000000000, 0.000000000000000000, -1.000000000000000000 ) ) ;
#101415=CARTESIAN_POINT ( 'NONE',  ( 1.649999999999949729, 2.500000000000000000, 5.902370205355745192 ) ) ;
#101417=DIRECTION ( 'NONE',  ( 0.000000000000000000, 1.000000000000000000, 0.000000000000000000 ) ) ;
#101418=EDGE_LOOP ( 'NONE', ( #16758, #50947 ) ) ;
#101419=VECTOR ( 'NONE', #39655, 1000.000000000000000 ) ;
#101420=AXIS2_PLACEMENT_3D ( 'NONE', #8995, #87559, #37826 ) ;
#101421=DIRECTION ( 'NONE',  ( 0.000000000000000000, 0.000000000000000000, 1.000000000000000000 ) ) ;
#101422=CARTESIAN_POINT ( 'NONE',  ( -6.650000000000018119, 2.500000000000000000, -6.595190528383302109 ) ) ;
#101423=ORIENTED_EDGE ( 'NONE', *, *, #29737, .T. ) ;
#101424=ORIENTED_EDGE ( 'NONE', *, *, #15292, .T. ) ;
#101425=FACE_OUTER_BOUND ( 'NONE', #15127, .T. ) ;
#101426=PLANE ( 'NONE',  #10987 ) ;
#101427=FACE_BOUND ( 'NONE', #14642, .T. ) ;
#101428=DIRECTION ( 'NONE',  ( -0.000000000000000000, 1.000000000000000000, -0.000000000000000000 ) ) ;
#101429=EDGE_CURVE ( 'NONE', #1020, #54054, #14731, .T. ) ;
#101430=VERTEX_POINT ( 'NONE', #114246 ) ;
#101431=DIRECTION ( 'NONE',  ( 0.000000000000000000, 0.000000000000000000, 1.000000000000000000 ) ) ;
#101432=EDGE_CURVE ( 'NONE', #25321, #68325, #55336, .T. ) ;
#101434=EDGE_CURVE ( 'NONE', #67249, #77153, #25065, .T. ) ;
#101435=EDGE_CURVE ( 'NONE', #55449, #7001, #43867, .T. ) ;
#101436=EDGE_LOOP ( 'NONE', ( #15789, #92790, #44952, #71785 ) ) ;
#101437=DIRECTION ( 'NONE',  ( 0.000000000000000000, 0.000000000000000000, -1.000000000000000000 ) ) ;
#101438=DIRECTION ( 'NONE',  ( 0.000000000000000000, 1.000000000000000000, 0.000000000000000000 ) ) ;
#101439=AXIS2_PLACEMENT_3D ( 'NONE', #27839, #65824, #87395 ) ;
#101440=CONICAL_SURFACE ( 'NONE', #38775, 0.1000000000000002554, 0.003490658503988666988 ) ;
#101441=ADVANCED_FACE ( 'NONE', ( #75596 ), #42966, .T. ) ;
#101442=ADVANCED_FACE ( 'NONE', ( #4919 ), #84786, .T. ) ;
#101443=CARTESIAN_POINT ( 'NONE',  ( -3.750000000000025757, 2.500000000000000000, -2.757883832488654097 ) ) ;
#101444=EDGE_CURVE ( 'NONE', #87657, #106953, #124713, .T. ) ;
#101445=CARTESIAN_POINT ( 'NONE',  ( 11.44999999999990514, 2.500000000000000000, -6.148780366869526226 ) ) ;
#101446=ORIENTED_EDGE ( 'NONE', *, *, #75435, .T. ) ;
#101447=DIRECTION ( 'NONE',  ( 0.000000000000000000, 0.000000000000000000, -1.000000000000000000 ) ) ;
#101448=EDGE_CURVE ( 'NONE', #122865, #8533, #74326, .T. ) ;
#101449=CARTESIAN_POINT ( 'NONE',  ( 10.64999999999991331, 2.500000000000000000, 6.048780366869521252 ) ) ;
#101450=DIRECTION ( 'NONE',  ( 0.000000000000000000, 0.000000000000000000, 1.000000000000000000 ) ) ;
#101451=ORIENTED_EDGE ( 'NONE', *, *, #27743, .T. ) ;
#101452=EDGE_LOOP ( 'NONE', ( #60207, #45915 ) ) ;
#101453=EDGE_CURVE ( 'NONE', #67694, #73914, #114930, .T. ) ;
#101454=DIRECTION ( 'NONE',  ( 0.000000000000000000, 0.000000000000000000, 1.000000000000000000 ) ) ;
#101455=VECTOR ( 'NONE', #3286, 1000.000000000000000 ) ;
#101456=EDGE_CURVE ( 'NONE', #93396, #34419, #94590, .T. ) ;
#101457=ORIENTED_EDGE ( 'NONE', *, *, #88953, .T. ) ;
#101458=DIRECTION ( 'NONE',  ( 0.000000000000000000, 0.000000000000000000, 1.000000000000000000 ) ) ;
#101459=DIRECTION ( 'NONE',  ( 0.000000000000000000, 1.000000000000000000, 0.000000000000000000 ) ) ;
#101460=AXIS2_PLACEMENT_3D ( 'NONE', #1621, #50730, #81488 ) ;
#101461=CARTESIAN_POINT ( 'NONE',  ( -1.650000000000034328, 12.50000000000000000, -7.253104124594891289 ) ) ;
#101462=VERTEX_POINT ( 'NONE', #4268 ) ;
#101463=CIRCLE ( 'NONE', #93061, 0.06509327318403745899 ) ;
#101464=DIRECTION ( 'NONE',  ( 0.000000000000000000, 0.000000000000000000, 1.000000000000000000 ) ) ;
#101465=DIRECTION ( 'NONE',  ( 0.000000000000000000, 0.000000000000000000, 1.000000000000000000 ) ) ;
#101466=CARTESIAN_POINT ( 'NONE',  ( -13.09999999999999254, 2.500000000000000000, -3.983716857408423628 ) ) ;
#101467=AXIS2_PLACEMENT_3D ( 'NONE', #55104, #125747, #124495 ) ;
#101468=DIRECTION ( 'NONE',  ( -4.274815082592931898E-19, -0.9999939076577903929, -0.003490651415223739937 ) ) ;
#101470=CARTESIAN_POINT ( 'NONE',  ( 6.449999999999930012, 2.500000000000000000, 1.718653347947321386 ) ) ;
#101471=AXIS2_PLACEMENT_3D ( 'NONE', #103603, #124531, #25665 ) ;
#101472=ORIENTED_EDGE ( 'NONE', *, *, #60269, .F. ) ;
#101473=AXIS2_PLACEMENT_3D ( 'NONE', #41113, #81653, #101948 ) ;
#101474=ORIENTED_EDGE ( 'NONE', *, *, #36165, .F. ) ;
#101475=CIRCLE ( 'NONE', #28312, 0.06509327318403745899 ) ;
#101476=CARTESIAN_POINT ( 'NONE',  ( 1.649999999999949729, 12.50000000000000000, 7.188010851410848723 ) ) ;
#101477=ORIENTED_EDGE ( 'NONE', *, *, #92621, .T. ) ;
#101478=LINE ( 'NONE', #3906, #124599 ) ;
#101480=VERTEX_POINT ( 'NONE', #44209 ) ;
#101481=ORIENTED_EDGE ( 'NONE', *, *, #63015, .T. ) ;
#101482=EDGE_LOOP ( 'NONE', ( #100393, #12753 ) ) ;
#101483=DIRECTION ( 'NONE',  ( -0.000000000000000000, 1.000000000000000000, -0.000000000000000000 ) ) ;
#101484=CIRCLE ( 'NONE', #88861, 0.06509327318403745899 ) ;
#101485=CARTESIAN_POINT ( 'NONE',  ( 9.799999999999913669, 2.500000000000000000, -3.983716857408426293 ) ) ;
#101486=AXIS2_PLACEMENT_3D ( 'NONE', #31587, #74082, #42719 ) ;
#101487=FACE_OUTER_BOUND ( 'NONE', #28388, .T. ) ;
#101488=VECTOR ( 'NONE', #35484, 1000.000000000000000 ) ;
#101489=DIRECTION ( 'NONE',  ( 0.000000000000000000, 0.000000000000000000, 1.000000000000000000 ) ) ;
#101490=CARTESIAN_POINT ( 'NONE',  ( 3.349999999999945466, 2.500000000000000000, -2.857883832488653741 ) ) ;
#101491=DIRECTION ( 'NONE',  ( -0.000000000000000000, -1.000000000000000000, -0.000000000000000000 ) ) ;
#101492=CONICAL_SURFACE ( 'NONE', #57663, 0.1000000000000000056, 0.003490658503988666988 ) ;
#101493=CARTESIAN_POINT ( 'NONE',  ( -6.450000000000016165, 2.500000000000000000, 2.511473670974873507 ) ) ;
#101494=DIRECTION ( 'NONE',  ( 0.000000000000000000, -0.9999939076577903929, 0.003490651415223739937 ) ) ;
#101495=CARTESIAN_POINT ( 'NONE',  ( 0.3999999999999568345, 2.500000000000000000, -3.737306695894649700 ) ) ;
#101496=ORIENTED_EDGE ( 'NONE', *, *, #16989, .T. ) ;
#101497=EDGE_CURVE ( 'NONE', #5264, #70467, #58534, .T. ) ;
#101498=EDGE_CURVE ( 'NONE', #81764, #44564, #48062, .T. ) ;
#101499=DIRECTION ( 'NONE',  ( 0.000000000000000000, 0.000000000000000000, -1.000000000000000000 ) ) ;
#101500=EDGE_LOOP ( 'NONE', ( #108003, #22852 ) ) ;
#101501=ORIENTED_EDGE ( 'NONE', *, *, #19659, .F. ) ;
#101502=DIRECTION ( 'NONE',  ( 0.000000000000000000, 0.000000000000000000, 1.000000000000000000 ) ) ;
#101503=DIRECTION ( 'NONE',  ( 0.000000000000000000, 0.000000000000000000, 1.000000000000000000 ) ) ;
#101504=CIRCLE ( 'NONE', #122435, 0.06509327318403745899 ) ;
#101505=CARTESIAN_POINT ( 'NONE',  ( -11.44999999999999751, 2.500000000000000000, 6.248780366869521430 ) ) ;
#101506=CARTESIAN_POINT ( 'NONE',  ( 10.39999999999991509, 12.50000000000000000, -0.6277270498435167934 ) ) ;
#101507=CARTESIAN_POINT ( 'NONE',  ( -5.400000000000024336, 2.500000000000000000, -3.537306695894649966 ) ) ;
#101508=B_SPLINE_SURFACE_WITH_KNOTS ( 'NONE', 3, 1, ( 
 ( #96283, #46542 ),
 ( #86470, #126406 ),
 ( #36754, #76663 ),
 ( #77943, #19008 ),
 ( #68763, #60267 ),
 ( #118507, #98223 ),
 ( #39966, #40629 ),
 ( #109338, #79250 ),
 ( #49795, #97581 ),
 ( #38695, #79880 ),
 ( #80536, #120451 ),
 ( #119804, #69403 ),
 ( #47857, #30801 ),
 ( #88391, #25 ),
 ( #17719, #87753 ),
 ( #70703, #57673 ),
 ( #18373, #29499 ),
 ( #58958, #89699 ) ),
 .UNSPECIFIED., .F., .F., .F.,
 ( 4, 2, 2, 2, 2, 2, 2, 2, 4 ),
 ( 2, 2 ),
 ( 0.000000000000000000, 0.1250000000000000000, 0.2500000000000000000, 0.3750000000000000000, 0.5000000000000000000, 0.6250000000000000000, 0.7500000000000000000, 0.8750000000000000000, 1.000000000000000000 ),
 ( 0.000000000000000000, 1.000000000000000000 ),
 .UNSPECIFIED. ) ;
#101509=DIRECTION ( 'NONE',  ( -0.000000000000000000, -1.000000000000000000, -0.000000000000000000 ) ) ;
#101510=PLANE ( 'NONE',  #69814 ) ;
#101511=EDGE_LOOP ( 'NONE', ( #118269, #33907, #45507, #58744 ) ) ;
#101512=AXIS2_PLACEMENT_3D ( 'NONE', #4037, #5963, #105476 ) ;
#101513=CIRCLE ( 'NONE', #120292, 0.06509327318403745899 ) ;
#101514=AXIS2_PLACEMENT_3D ( 'NONE', #47500, #7551, #97234 ) ;
#101515=EDGE_LOOP ( 'NONE', ( #72917, #55387, #126677, #79019 ) ) ;
#101516=VERTEX_POINT ( 'NONE', #97188 ) ;
#101517=ORIENTED_EDGE ( 'NONE', *, *, #48973, .F. ) ;
#101518=ORIENTED_EDGE ( 'NONE', *, *, #110324, .T. ) ;
#101519=DIRECTION ( 'NONE',  ( -4.274815082592931898E-19, -0.9999939076577903929, -0.003490651415223739937 ) ) ;
#101520=DIRECTION ( 'NONE',  ( 0.000000000000000000, 0.000000000000000000, 1.000000000000000000 ) ) ;
#101521=VECTOR ( 'NONE', #57619, 1000.000000000000000 ) ;
#101522=DIRECTION ( 'NONE',  ( 0.000000000000000000, 0.000000000000000000, 1.000000000000000000 ) ) ;
#101523=DIRECTION ( 'NONE',  ( 0.000000000000000000, 0.000000000000000000, 1.000000000000000000 ) ) ;
#101524=CIRCLE ( 'NONE', #42971, 0.1000000000000000472 ) ;
#101525=FACE_OUTER_BOUND ( 'NONE', #81813, .T. ) ;
#101526=ORIENTED_EDGE ( 'NONE', *, *, #108527, .F. ) ;
#101527=PLANE ( 'NONE',  #20661 ) ;
#101528=DIRECTION ( 'NONE',  ( 0.000000000000000000, 0.000000000000000000, 1.000000000000000000 ) ) ;
#101529=DIRECTION ( 'NONE',  ( -0.000000000000000000, 1.000000000000000000, -0.000000000000000000 ) ) ;
#101530=DIRECTION ( 'NONE',  ( 0.000000000000000000, -0.000000000000000000, 1.000000000000000000 ) ) ;
#101531=CARTESIAN_POINT ( 'NONE',  ( -1.650000000000034328, 12.50000000000000000, -7.188010851410854052 ) ) ;
#101532=EDGE_CURVE ( 'NONE', #84837, #92462, #121201, .T. ) ;
#101533=ORIENTED_EDGE ( 'NONE', *, *, #128490, .T. ) ;
#101534=CIRCLE ( 'NONE', #17894, 0.1000000000000002554 ) ;
#101535=CIRCLE ( 'NONE', #5378, 0.09999999999999982514 ) ;
#101536=ORIENTED_EDGE ( 'NONE', *, *, #72801, .F. ) ;
#101537=VERTEX_POINT ( 'NONE', #125985 ) ;
#101538=CARTESIAN_POINT ( 'NONE',  ( -3.100000000000028955, 2.500000000000000000, 4.776537180435972196 ) ) ;
#101539=ORIENTED_EDGE ( 'NONE', *, *, #111957, .F. ) ;
#101540=DIRECTION ( 'NONE',  ( -4.274815082592931898E-19, -0.9999939076577903929, -0.003490651415223739937 ) ) ;
#101541=DIRECTION ( 'NONE',  ( 0.000000000000000000, 0.000000000000000000, 1.000000000000000000 ) ) ;
#101542=ADVANCED_FACE ( 'NONE', ( #57267 ), #106531, .T. ) ;
#101543=EDGE_CURVE ( 'NONE', #128383, #106389, #64766, .T. ) ;
#101544=ORIENTED_EDGE ( 'NONE', *, *, #46690, .F. ) ;
#101546=DIRECTION ( 'NONE',  ( 0.000000000000000000, 0.000000000000000000, -1.000000000000000000 ) ) ;
#101547=LINE ( 'NONE', #20413, #115100 ) ;
#101548=EDGE_CURVE ( 'NONE', #55365, #110679, #71039, .T. ) ;
#101549=CARTESIAN_POINT ( 'NONE',  ( -11.44999999999999929, 2.500000000000000000, -6.048780366869523029 ) ) ;
#101550=VECTOR ( 'NONE', #12580, 1000.000000000000000 ) ;
#101551=CARTESIAN_POINT ( 'NONE',  ( -13.14999999999999147, 2.500000000000000000, -1.818653347947323917 ) ) ;
#101552=EDGE_CURVE ( 'NONE', #32372, #94402, #46148, .T. ) ;
#101553=AXIS2_PLACEMENT_3D ( 'NONE', #6664, #56435, #93803 ) ;
#101554=ORIENTED_EDGE ( 'NONE', *, *, #43832, .T. ) ;
#101556=ORIENTED_EDGE ( 'NONE', *, *, #9143, .T. ) ;
#101557=EDGE_CURVE ( 'NONE', #102950, #117733, #83567, .T. ) ;
#101558=LINE ( 'NONE', #33471, #64730 ) ;
#101559=CARTESIAN_POINT ( 'NONE',  ( -13.74999999999998934, 2.500000000000000000, 2.957883832488652942 ) ) ;
#101560=DIRECTION ( 'NONE',  ( -0.000000000000000000, 1.000000000000000000, -0.000000000000000000 ) ) ;
#101561=DIRECTION ( 'NONE',  ( 0.000000000000000000, 0.000000000000000000, -1.000000000000000000 ) ) ;
#101562=VERTEX_POINT ( 'NONE', #126654 ) ;
#101563=CIRCLE ( 'NONE', #124559, 0.1000000000000002554 ) ;
#101565=DIRECTION ( 'NONE',  ( -4.274815082592931898E-19, -0.9999939076577903929, -0.003490651415223739937 ) ) ;
#101566=DIRECTION ( 'NONE',  ( 0.000000000000000000, 1.000000000000000000, 0.000000000000000000 ) ) ;
#101567=DIRECTION ( 'NONE',  ( 0.000000000000000000, -0.000000000000000000, 1.000000000000000000 ) ) ;
#101568=FACE_OUTER_BOUND ( 'NONE', #73544, .T. ) ;
#101569=VERTEX_POINT ( 'NONE', #128615 ) ;
#101571=CIRCLE ( 'NONE', #118286, 0.09999999999999982514 ) ;
#101572=DIRECTION ( 'NONE',  ( 0.000000000000000000, 0.000000000000000000, 1.000000000000000000 ) ) ;
#101573=FACE_OUTER_BOUND ( 'NONE', #118871, .T. ) ;
#101574=AXIS2_PLACEMENT_3D ( 'NONE', #119080, #11038, #52275 ) ;
#101576=DIRECTION ( 'NONE',  ( -0.000000000000000000, 1.000000000000000000, -0.000000000000000000 ) ) ;
#101577=EDGE_LOOP ( 'NONE', ( #99679, #32553, #39399, #36504 ) ) ;
#101578=CARTESIAN_POINT ( 'NONE',  ( -6.650000000000015454, 2.500000000000000000, 7.088010851410848190 ) ) ;
#101579=ORIENTED_EDGE ( 'NONE', *, *, #12176, .F. ) ;
#101580=ADVANCED_FACE ( 'NONE', ( #78859 ), #87739, .T. ) ;
#101581=ORIENTED_EDGE ( 'NONE', *, *, #36344, .T. ) ;
#101582=DIRECTION ( 'NONE',  ( -0.000000000000000000, -1.000000000000000000, -0.000000000000000000 ) ) ;
#101583=DIRECTION ( 'NONE',  ( -0.000000000000000000, -1.000000000000000000, -0.000000000000000000 ) ) ;
#101584=EDGE_LOOP ( 'NONE', ( #9661, #74054, #88160, #21811 ) ) ;
#101585=EDGE_LOOP ( 'NONE', ( #46850, #88351 ) ) ;
#101586=EDGE_CURVE ( 'NONE', #53470, #101913, #29113, .T. ) ;
#101587=CARTESIAN_POINT ( 'NONE',  ( -11.24999999999996447, 2.500000000000000000, -2.265063509461097802 ) ) ;
#101589=AXIS2_PLACEMENT_3D ( 'NONE', #81789, #32082, #71998 ) ;
#101590=EDGE_CURVE ( 'NONE', #94018, #35080, #116815, .T. ) ;
#101591=DIRECTION ( 'NONE',  ( 0.000000000000000000, 0.000000000000000000, -1.000000000000000000 ) ) ;
#101593=DIRECTION ( 'NONE',  ( 0.000000000000000000, 1.000000000000000000, 0.000000000000000000 ) ) ;
#101595=CARTESIAN_POINT ( 'NONE',  ( 9.999999999999914735, 12.50000000000000000, 0.6928203230275494784 ) ) ;
#101596=EDGE_CURVE ( 'NONE', #65177, #34926, #18791, .T. ) ;
#101597=ADVANCED_FACE ( 'NONE', ( #57920 ), #125411, .T. ) ;
#101598=DIRECTION ( 'NONE',  ( -0.000000000000000000, -1.000000000000000000, -0.000000000000000000 ) ) ;
#101600=CARTESIAN_POINT ( 'NONE',  ( -11.05000000000000071, 12.50000000000000000, -2.511473670974873951 ) ) ;
#101601=ADVANCED_FACE ( 'NONE', ( #27155 ), #29279, .T. ) ;
#101602=CIRCLE ( 'NONE', #22294, 0.06509327318403743123 ) ;
#101603=EDGE_CURVE ( 'NONE', #31883, #45092, #85696, .T. ) ;
#101604=AXIS2_PLACEMENT_3D ( 'NONE', #111567, #120741, #21245 ) ;
#101605=VERTEX_POINT ( 'NONE', #8791 ) ;
#101606=CIRCLE ( 'NONE', #17968, 0.1000000000000002554 ) ;
#101607=ORIENTED_EDGE ( 'NONE', *, *, #104284, .T. ) ;
#101608=DIRECTION ( 'NONE',  ( 0.000000000000000000, 1.000000000000000000, 0.000000000000000000 ) ) ;
#101609=EDGE_CURVE ( 'NONE', #108744, #104158, #6839, .T. ) ;
#101610=EDGE_LOOP ( 'NONE', ( #124414, #42867, #116296, #89971 ) ) ;
#101611=DIRECTION ( 'NONE',  ( 0.000000000000000000, 0.000000000000000000, -1.000000000000000000 ) ) ;
#101612=CARTESIAN_POINT ( 'NONE',  ( -8.750000000000010658, 2.500000000000000000, 2.857883832488649301 ) ) ;
#101613=DIRECTION ( 'NONE',  ( 0.000000000000000000, 1.000000000000000000, 0.000000000000000000 ) ) ;
#101614=EDGE_LOOP ( 'NONE', ( #107397, #77114 ) ) ;
#101615=ORIENTED_EDGE ( 'NONE', *, *, #92411, .F. ) ;
#101616=FACE_BOUND ( 'NONE', #48249, .T. ) ;
#101617=ORIENTED_EDGE ( 'NONE', *, *, #111016, .T. ) ;
#101618=DIRECTION ( 'NONE',  ( 0.000000000000000000, 0.000000000000000000, -1.000000000000000000 ) ) ;
#101619=CARTESIAN_POINT ( 'NONE',  ( -7.300000000000016698, 2.500000000000000000, -4.676537180435978769 ) ) ;
#101620=EDGE_CURVE ( 'NONE', #72103, #57756, #119147, .T. ) ;
#101621=AXIS2_PLACEMENT_3D ( 'NONE', #40417, #69194, #118308 ) ;
#101622=DIRECTION ( 'NONE',  ( -4.274815082592931898E-19, -0.9999939076577903929, -0.003490651415223739937 ) ) ;
#101623=DIRECTION ( 'NONE',  ( 0.000000000000000000, 0.000000000000000000, -1.000000000000000000 ) ) ;
#101624=CARTESIAN_POINT ( 'NONE',  ( 10.79999999999991012, 2.500000000000000000, -4.430127018922202176 ) ) ;
#101625=AXIS2_PLACEMENT_3D ( 'NONE', #6449, #55591, #57533 ) ;
#101626=CONICAL_SURFACE ( 'NONE', #9670, 0.1000000000000000472, 0.003490658503988666988 ) ;
#101627=CARTESIAN_POINT ( 'NONE',  ( 9.149999999999915090, 12.50000000000000000, 6.560283801567334372 ) ) ;
#101628=CARTESIAN_POINT ( 'NONE',  ( 1.649999999999951950, 2.500000000000000000, -5.802370205355749988 ) ) ;
#101629=FACE_OUTER_BOUND ( 'NONE', #120234, .T. ) ;
#101630=CARTESIAN_POINT ( 'NONE',  ( 11.69999999999990514, 2.500000000000000000, 0.09999999999999772959 ) ) ;
#101631=CARTESIAN_POINT ( 'NONE',  ( 9.549999999999915445, 2.500000000000000000, 6.595190528383296780 ) ) ;
#101632=DIRECTION ( 'NONE',  ( -4.274815082592931898E-19, -0.9999939076577903929, -0.003490651415223739937 ) ) ;
#101633=ORIENTED_EDGE ( 'NONE', *, *, #112188, .F. ) ;
#101635=ORIENTED_EDGE ( 'NONE', *, *, #107523, .T. ) ;
#101637=CARTESIAN_POINT ( 'NONE',  ( 12.49999999999990408, 12.50000000000000000, 5.088040615133786027 ) ) ;
#101638=DIRECTION ( 'NONE',  ( 0.000000000000000000, -0.9999939076577903929, 0.003490651415223739937 ) ) ;
#101639=ORIENTED_EDGE ( 'NONE', *, *, #78989, .T. ) ;
#101640=ORIENTED_EDGE ( 'NONE', *, *, #115704, .F. ) ;
#101641=EDGE_LOOP ( 'NONE', ( #123659, #47851, #129579, #105139 ) ) ;
#101642=LINE ( 'NONE', #123830, #29255 ) ;
#101643=CARTESIAN_POINT ( 'NONE',  ( -2.500000000000030642, 2.500000000000000000, -0.5928203230275541635 ) ) ;
#101644=CARTESIAN_POINT ( 'NONE',  ( 12.89999999999990088, 12.50000000000000000, 4.330127018922196314 ) ) ;
#101645=DIRECTION ( 'NONE',  ( 0.000000000000000000, 1.000000000000000000, 0.000000000000000000 ) ) ;
#101646=CARTESIAN_POINT ( 'NONE',  ( -0.4000000000000396572, 2.500000000000000000, 4.230127018922196669 ) ) ;
#101647=CARTESIAN_POINT ( 'NONE',  ( -1.900000000000034106, 2.500000000000000000, 0.3464101615137735735 ) ) ;
#101648=ADVANCED_FACE ( 'NONE', ( #47448 ), #96242, .T. ) ;
#101649=ORIENTED_EDGE ( 'NONE', *, *, #113177, .F. ) ;
#101650=DIRECTION ( 'NONE',  ( 0.000000000000000000, 1.000000000000000000, 0.000000000000000000 ) ) ;
#101651=ORIENTED_EDGE ( 'NONE', *, *, #27775, .T. ) ;
#101652=AXIS2_PLACEMENT_3D ( 'NONE', #113366, #45291, #74740 ) ;
#101653=VERTEX_POINT ( 'NONE', #118108 ) ;
#101655=ORIENTED_EDGE ( 'NONE', *, *, #79518, .F. ) ;
#101656=VECTOR ( 'NONE', #107485, 1000.000000000000000 ) ;
#101658=VERTEX_POINT ( 'NONE', #79493 ) ;
#101659=EDGE_LOOP ( 'NONE', ( #277, #25139, #89860, #60824 ) ) ;
#101660=ORIENTED_EDGE ( 'NONE', *, *, #3121, .T. ) ;
#101661=CARTESIAN_POINT ( 'NONE',  ( 9.549999999999915445, 12.50000000000000000, -2.099970236277064473 ) ) ;
#101662=AXIS2_PLACEMENT_3D ( 'NONE', #86718, #38943, #99126 ) ;
#101663=ADVANCED_FACE ( 'NONE', ( #61132 ), #79540, .T. ) ;
#101664=DIRECTION ( 'NONE',  ( 0.000000000000000000, 0.000000000000000000, -1.000000000000000000 ) ) ;
#101665=CARTESIAN_POINT ( 'NONE',  ( -14.14999999999998614, 2.500000000000000000, 1.572243186433549544 ) ) ;
#101666=CARTESIAN_POINT ( 'NONE',  ( -4.800000000000028244, 2.500000000000000000, -3.983716857408426293 ) ) ;
#101667=FACE_OUTER_BOUND ( 'NONE', #73445, .T. ) ;
#101668=DIRECTION ( 'NONE',  ( 0.000000000000000000, 1.000000000000000000, 0.000000000000000000 ) ) ;
#101669=CARTESIAN_POINT ( 'NONE',  ( -11.05000000000000071, 2.500000000000000000, -2.611473670974873595 ) ) ;
#101670=AXIS2_PLACEMENT_3D ( 'NONE', #15200, #3476, #103622 ) ;
#101671=AXIS2_PLACEMENT_3D ( 'NONE', #59738, #17847, #57788 ) ;
#101672=EDGE_LOOP ( 'NONE', ( #64611, #76391, #110966, #40049 ) ) ;
#101673=DIRECTION ( 'NONE',  ( -0.000000000000000000, 1.000000000000000000, -0.000000000000000000 ) ) ;
#101674=AXIS2_PLACEMENT_3D ( 'NONE', #22929, #62217, #43226 ) ;
#101675=VERTEX_POINT ( 'NONE', #82049 ) ;
#101676=FACE_OUTER_BOUND ( 'NONE', #72555, .T. ) ;
#101677=VERTEX_POINT ( 'NONE', #31052 ) ;
#101678=CARTESIAN_POINT ( 'NONE',  ( 8.949999999999921130, 2.500000000000000000, 1.718653347947321386 ) ) ;
#101679=EDGE_LOOP ( 'NONE', ( #86372, #4478, #27978, #86265 ) ) ;
#101680=CARTESIAN_POINT ( 'NONE',  ( 3.349999999999945466, 12.50000000000000000, -6.495190528383302464 ) ) ;
#101681=CARTESIAN_POINT ( 'NONE',  ( -6.650000000000018119, 2.500000000000000000, -7.288010851410854585 ) ) ;
#101682=ORIENTED_EDGE ( 'NONE', *, *, #28316, .T. ) ;
#101683=ORIENTED_EDGE ( 'NONE', *, *, #22987, .F. ) ;
#101684=FACE_OUTER_BOUND ( 'NONE', #25766, .T. ) ;
#101685=CARTESIAN_POINT ( 'NONE',  ( 4.149999999999939959, 2.500000000000000000, 1.472243186433545459 ) ) ;
#101686=LINE ( 'NONE', #129239, #68885 ) ;
#101687=AXIS2_PLACEMENT_3D ( 'NONE', #46377, #86299, #36597 ) ;
#101688=DIRECTION ( 'NONE',  ( -0.000000000000000000, 1.000000000000000000, -0.000000000000000000 ) ) ;
#101689=CARTESIAN_POINT ( 'NONE',  ( -9.200000000000009948, 2.500000000000000000, -4.430127018922197735 ) ) ;
#101690=ORIENTED_EDGE ( 'NONE', *, *, #108666, .F. ) ;
#101691=CONICAL_SURFACE ( 'NONE', #78712, 0.1000000000000000472, 0.003490658503988666988 ) ;
#101693=DIRECTION ( 'NONE',  ( 0.000000000000000000, -0.9999939076577903929, 0.003490651415223739937 ) ) ;
#101694=AXIS2_PLACEMENT_3D ( 'NONE', #96135, #9036, #47696 ) ;
#101695=AXIS2_PLACEMENT_3D ( 'NONE', #45897, #118335, #74705 ) ;
#101696=ORIENTED_EDGE ( 'NONE', *, *, #40689, .F. ) ;
#101697=VECTOR ( 'NONE', #106886, 1000.000000000000000 ) ;
#101698=PLANE ( 'NONE',  #17214 ) ;
#101700=EDGE_CURVE ( 'NONE', #55696, #9421, #75321, .T. ) ;
#101701=AXIS2_PLACEMENT_3D ( 'NONE', #65348, #124931, #117016 ) ;
#101702=ADVANCED_FACE ( 'NONE', ( #99129 ), #112980, .T. ) ;
#101703=ADVANCED_FACE ( 'NONE', ( #121988 ), #18887, .T. ) ;
#101704=DIRECTION ( 'NONE',  ( -4.274815082592931898E-19, -0.9999939076577903929, -0.003490651415223739937 ) ) ;
#101706=DIRECTION ( 'NONE',  ( 0.000000000000000000, 0.000000000000000000, 1.000000000000000000 ) ) ;
#101708=ADVANCED_FACE ( 'NONE', ( #21201 ), #115024, .T. ) ;
#101710=VERTEX_POINT ( 'NONE', #109594 ) ;
#101711=AXIS2_PLACEMENT_3D ( 'NONE', #41702, #64373, #61978 ) ;
#101713=AXIS2_PLACEMENT_3D ( 'NONE', #102592, #54779, #114351 ) ;
#101714=CIRCLE ( 'NONE', #97500, 0.06509327318403745899 ) ;
#101715=CARTESIAN_POINT ( 'NONE',  ( 4.349999999999939249, 12.50000000000000000, 2.511473670974873507 ) ) ;
#101716=CARTESIAN_POINT ( 'NONE',  ( -9.600000000000008527, 2.500000000000000000, 0.09999999999999761857 ) ) ;
#101717=EDGE_CURVE ( 'NONE', #113506, #76961, #64853, .T. ) ;
#101718=ORIENTED_EDGE ( 'NONE', *, *, #26216, .T. ) ;
#101720=ORIENTED_EDGE ( 'NONE', *, *, #87357, .T. ) ;
#101721=CARTESIAN_POINT ( 'NONE',  ( -5.850000000000018296, 2.500000000000000000, 7.188010851410848723 ) ) ;
#101722=VERTEX_POINT ( 'NONE', #50050 ) ;
#101723=ORIENTED_EDGE ( 'NONE', *, *, #53279, .T. ) ;
#101724=CARTESIAN_POINT ( 'NONE',  ( -13.74999999999998934, 2.500000000000000000, -1.472243186433547901 ) ) ;
#101725=ORIENTED_EDGE ( 'NONE', *, *, #68146, .F. ) ;
#101726=CARTESIAN_POINT ( 'NONE',  ( -1.850000000000033840, 12.50000000000000000, 2.446380397790835826 ) ) ;
#101727=DIRECTION ( 'NONE',  ( -0.000000000000000000, 1.000000000000000000, -0.000000000000000000 ) ) ;
#101728=CARTESIAN_POINT ( 'NONE',  ( 16.84158739990463616, 0.4722467112504742937, 5.802037699229681600 ) ) ;
#101729=ORIENTED_EDGE ( 'NONE', *, *, #12566, .T. ) ;
#101730=CARTESIAN_POINT ( 'NONE',  ( -14.34999999999998543, 2.500000000000000000, 2.511473670974877503 ) ) ;
#101731=DIRECTION ( 'NONE',  ( -0.000000000000000000, -1.000000000000000000, -0.000000000000000000 ) ) ;
#101732=ORIENTED_EDGE ( 'NONE', *, *, #91041, .T. ) ;
#101733=AXIS2_PLACEMENT_3D ( 'NONE', #90331, #677, #40640 ) ;
#101734=EDGE_LOOP ( 'NONE', ( #33153, #124008 ) ) ;
#101735=CIRCLE ( 'NONE', #62033, 0.1000000000000000472 ) ;
#101736=ORIENTED_EDGE ( 'NONE', *, *, #62556, .F. ) ;
#101737=CARTESIAN_POINT ( 'NONE',  ( 2.099999999999948574, 12.50000000000000000, 4.330127018922196314 ) ) ;
#101738=DIRECTION ( 'NONE',  ( 0.000000000000000000, 0.000000000000000000, 1.000000000000000000 ) ) ;
#101739=DIRECTION ( 'NONE',  ( 0.000000000000000000, -0.000000000000000000, 1.000000000000000000 ) ) ;
#101740=FACE_BOUND ( 'NONE', #126316, .T. ) ;
#101741=ORIENTED_EDGE ( 'NONE', *, *, #1542, .T. ) ;
#101742=DIRECTION ( 'NONE',  ( 0.000000000000000000, 0.000000000000000000, -1.000000000000000000 ) ) ;
#101743=CARTESIAN_POINT ( 'NONE',  ( 8.549999999999924327, 2.500000000000000000, -6.941600689897077459 ) ) ;
#101744=ORIENTED_EDGE ( 'NONE', *, *, #112275, .F. ) ;
#101745=VECTOR ( 'NONE', #113942, 1000.000000000000000 ) ;
#101746=CONICAL_SURFACE ( 'NONE', #126793, 0.1000000000000000472, 0.003490658503988666988 ) ;
#101747=CARTESIAN_POINT ( 'NONE',  ( 0.8499999999999536815, 2.500000000000000000, 5.802370205355744659 ) ) ;
#101748=DIRECTION ( 'NONE',  ( -0.000000000000000000, -1.000000000000000000, -0.000000000000000000 ) ) ;
#101749=CARTESIAN_POINT ( 'NONE',  ( 2.499999999999948930, 2.500000000000000000, -0.7928203230275542301 ) ) ;
#101750=ADVANCED_FACE ( 'NONE', ( #89936 ), #69061, .T. ) ;
#101751=CARTESIAN_POINT ( 'NONE',  ( 9.799999999999915445, 12.50000000000000000, 3.983716857408420964 ) ) ;
#101752=CARTESIAN_POINT ( 'NONE',  ( 2.899999999999946620, 2.500000000000000000, -3.637306695894650055 ) ) ;
#101753=EDGE_CURVE ( 'NONE', #59442, #31405, #23105, .T. ) ;
#101754=FACE_OUTER_BOUND ( 'NONE', #73946, .T. ) ;
#101755=CARTESIAN_POINT ( 'NONE',  ( -4.550000000000022915, 2.500000000000000000, 2.265063509461097357 ) ) ;
#101756=ADVANCED_FACE ( 'NONE', ( #40209 ), #71120, .T. ) ;
#101757=AXIS2_PLACEMENT_3D ( 'NONE', #79394, #106263, #108186 ) ;
#101758=VERTEX_POINT ( 'NONE', #40875 ) ;
#101759=ORIENTED_EDGE ( 'NONE', *, *, #50899, .F. ) ;
#101760=ADVANCED_FACE ( 'NONE', ( #120054 ), #123358, .T. ) ;
#101761=ORIENTED_EDGE ( 'NONE', *, *, #87631, .T. ) ;
#101762=EDGE_LOOP ( 'NONE', ( #44905, #40621, #77337, #16571 ) ) ;
#101763=CARTESIAN_POINT ( 'NONE',  ( 1.249999999999950262, 2.500000000000000000, 7.288010851410849256 ) ) ;
#101764=DIRECTION ( 'NONE',  ( -4.274815082592931898E-19, -0.9999939076577903929, -0.003490651415223739937 ) ) ;
#101766=FACE_BOUND ( 'NONE', #83553, .T. ) ;
#101767=DIRECTION ( 'NONE',  ( 0.000000000000000000, -0.000000000000000000, 1.000000000000000000 ) ) ;
#101768=DIRECTION ( 'NONE',  ( 0.000000000000000000, 0.000000000000000000, 1.000000000000000000 ) ) ;
#101769=ADVANCED_FACE ( 'NONE', ( #81426 ), #77390, .T. ) ;
#101770=CARTESIAN_POINT ( 'NONE',  ( -1.650000000000035660, 2.500000000000000000, 2.857883832488649301 ) ) ;
#101772=CARTESIAN_POINT ( 'NONE',  ( 9.199999999999915801, 12.50000000000000000, -4.330127018922201643 ) ) ;
#101773=DIRECTION ( 'NONE',  ( 0.000000000000000000, 0.000000000000000000, 1.000000000000000000 ) ) ;
#101774=DIRECTION ( 'NONE',  ( 0.000000000000000000, 0.000000000000000000, 1.000000000000000000 ) ) ;
#101775=DIRECTION ( 'NONE',  ( -0.000000000000000000, 1.000000000000000000, -0.000000000000000000 ) ) ;
#101776=DIRECTION ( 'NONE',  ( 0.000000000000000000, 0.000000000000000000, -1.000000000000000000 ) ) ;
#101777=DIRECTION ( 'NONE',  ( 0.000000000000000000, 1.000000000000000000, 0.000000000000000000 ) ) ;
#101778=AXIS2_PLACEMENT_3D ( 'NONE', #127386, #57349, #37715 ) ;
#101779=ORIENTED_EDGE ( 'NONE', *, *, #8141, .T. ) ;
#101780=VECTOR ( 'NONE', #96289, 1000.000000000000000 ) ;
#101782=AXIS2_PLACEMENT_3D ( 'NONE', #72171, #23059, #62979 ) ;
#101783=ORIENTED_EDGE ( 'NONE', *, *, #27117, .F. ) ;
#101785=AXIS2_PLACEMENT_3D ( 'NONE', #18491, #19115, #17173 ) ;
#101786=VERTEX_POINT ( 'NONE', #100414 ) ;
#101787=VERTEX_POINT ( 'NONE', #10711 ) ;
#101788=ORIENTED_EDGE ( 'NONE', *, *, #18579, .T. ) ;
#101789=ORIENTED_EDGE ( 'NONE', *, *, #8869, .T. ) ;
#101790=DIRECTION ( 'NONE',  ( 0.000000000000000000, 0.000000000000000000, 1.000000000000000000 ) ) ;
#101791=ORIENTED_EDGE ( 'NONE', *, *, #122283, .F. ) ;
#101792=CIRCLE ( 'NONE', #43305, 0.09999999999999982514 ) ;
#101793=EDGE_LOOP ( 'NONE', ( #24677, #90333, #122324, #125652 ) ) ;
#101794=CIRCLE ( 'NONE', #118492, 0.06509327318403745899 ) ;
#101795=CIRCLE ( 'NONE', #36951, 0.1000000000000000472 ) ;
#101796=DIRECTION ( 'NONE',  ( 0.000000000000000000, 0.000000000000000000, -1.000000000000000000 ) ) ;
#101797=CARTESIAN_POINT ( 'NONE',  ( -2.100000000000033396, 12.50000000000000000, -0.6277270498435167934 ) ) ;
#101798=CARTESIAN_POINT ( 'NONE',  ( 1.699999999999951994, 12.50000000000000000, -2.276824562219559311E-15 ) ) ;
#101799=DIRECTION ( 'NONE',  ( -0.000000000000000000, 1.000000000000000000, -0.000000000000000000 ) ) ;
#101800=CIRCLE ( 'NONE', #32853, 0.1000000000000002554 ) ;
#101801=ORIENTED_EDGE ( 'NONE', *, *, #29039, .F. ) ;
#101802=DIRECTION ( 'NONE',  ( 0.000000000000000000, -0.9999939076577903929, 0.003490651415223739937 ) ) ;
#101803=AXIS2_PLACEMENT_3D ( 'NONE', #24948, #53760, #102846 ) ;
#101804=ORIENTED_EDGE ( 'NONE', *, *, #42323, .T. ) ;
#101805=AXIS2_PLACEMENT_3D ( 'NONE', #123374, #101167, #21979 ) ;
#101806=CIRCLE ( 'NONE', #49580, 0.06509327318403745899 ) ;
#101807=ORIENTED_EDGE ( 'NONE', *, *, #46477, .F. ) ;
#101809=DIRECTION ( 'NONE',  ( -0.000000000000000000, -1.000000000000000000, -0.000000000000000000 ) ) ;
#101810=ORIENTED_EDGE ( 'NONE', *, *, #51003, .F. ) ;
#101811=ORIENTED_EDGE ( 'NONE', *, *, #128717, .F. ) ;
#101812=CARTESIAN_POINT ( 'NONE',  ( -3.750000000000027534, 2.500000000000000000, -1.572243186433550211 ) ) ;
#101813=ADVANCED_FACE ( 'NONE', ( #124570 ), #117078, .T. ) ;
#101814=DIRECTION ( 'NONE',  ( 0.000000000000000000, 1.000000000000000000, 0.000000000000000000 ) ) ;
#101815=PLANE ( 'NONE',  #12239 ) ;
#101816=DIRECTION ( 'NONE',  ( 0.000000000000000000, 0.000000000000000000, 1.000000000000000000 ) ) ;
#101817=PLANE ( 'NONE',  #123430 ) ;
#101818=VECTOR ( 'NONE', #32586, 1000.000000000000000 ) ;
#101819=VERTEX_POINT ( 'NONE', #23135 ) ;
#101820=LINE ( 'NONE', #42257, #126332 ) ;
#101821=EDGE_LOOP ( 'NONE', ( #96153, #115401, #5999, #42017 ) ) ;
#101823=CARTESIAN_POINT ( 'NONE',  ( -6.850000000000013856, 2.500000000000000000, 6.248780366869521430 ) ) ;
#101824=LINE ( 'NONE', #112927, #117988 ) ;
#101825=DIRECTION ( 'NONE',  ( 0.000000000000000000, 0.000000000000000000, -1.000000000000000000 ) ) ;
#101826=CARTESIAN_POINT ( 'NONE',  ( -9.350000000000008527, 12.50000000000000000, -6.841600689897072485 ) ) ;
#101827=VERTEX_POINT ( 'NONE', #73515 ) ;
#101828=FACE_OUTER_BOUND ( 'NONE', #52934, .T. ) ;
#101829=VECTOR ( 'NONE', #41828, 1000.000000000000000 ) ;
#101830=DIRECTION ( 'NONE',  ( 0.000000000000000000, 1.000000000000000000, 0.000000000000000000 ) ) ;
#101831=EDGE_LOOP ( 'NONE', ( #42316, #76835, #50080, #17628 ) ) ;
#101832=VERTEX_POINT ( 'NONE', #5419 ) ;
#101833=ORIENTED_EDGE ( 'NONE', *, *, #59893, .T. ) ;
#101834=CARTESIAN_POINT ( 'NONE',  ( 17.50000000000000000, 2.750000000000000000, 3.432456362931491700 ) ) ;
#101835=CARTESIAN_POINT ( 'NONE',  ( -10.20000000000000284, 2.500000000000000000, -0.2464101615137782308 ) ) ;
#101837=CARTESIAN_POINT ( 'NONE',  ( -5.850000000000019185, 2.500000000000000000, 2.265063509461097357 ) ) ;
#101838=AXIS2_PLACEMENT_3D ( 'NONE', #45846, #6518, #85753 ) ;
#101839=CARTESIAN_POINT ( 'NONE',  ( 9.999999999999916511, 12.50000000000000000, -0.6928203230275541413 ) ) ;
#101840=AXIS2_PLACEMENT_3D ( 'NONE', #53562, #92181, #93489 ) ;
#101841=CARTESIAN_POINT ( 'NONE',  ( 1.249999999999953815, 2.500000000000000000, 1.472243186433545459 ) ) ;
#101842=DIRECTION ( 'NONE',  ( 0.000000000000000000, 0.000000000000000000, 1.000000000000000000 ) ) ;
#101843=DIRECTION ( 'NONE',  ( 0.000000000000000000, 1.000000000000000000, 0.000000000000000000 ) ) ;
#101844=AXIS2_PLACEMENT_3D ( 'NONE', #22019, #121473, #10857 ) ;
#101845=AXIS2_PLACEMENT_3D ( 'NONE', #71300, #41867, #121053 ) ;
#101846=AXIS2_PLACEMENT_3D ( 'NONE', #81949, #20470, #818 ) ;
#101847=EDGE_CURVE ( 'NONE', #9468, #109985, #33490, .T. ) ;
#101848=ORIENTED_EDGE ( 'NONE', *, *, #59311, .T. ) ;
#101849=DIRECTION ( 'NONE',  ( -0.000000000000000000, 1.000000000000000000, -0.000000000000000000 ) ) ;
#101850=EDGE_CURVE ( 'NONE', #29463, #51752, #56540, .T. ) ;
#101851=FACE_OUTER_BOUND ( 'NONE', #30928, .T. ) ;
#101852=DIRECTION ( 'NONE',  ( 0.000000000000000000, 1.000000000000000000, 0.000000000000000000 ) ) ;
#101853=DIRECTION ( 'NONE',  ( 0.000000000000000000, 0.000000000000000000, 1.000000000000000000 ) ) ;
#101854=ADVANCED_FACE ( 'NONE', ( #4122 ), #29378, .T. ) ;
#101855=EDGE_LOOP ( 'NONE', ( #124770, #84468, #22745, #9459 ) ) ;
#101856=DIRECTION ( 'NONE',  ( -0.000000000000000000, 1.000000000000000000, -0.000000000000000000 ) ) ;
#101857=DIRECTION ( 'NONE',  ( -0.000000000000000000, -1.000000000000000000, -0.000000000000000000 ) ) ;
#101858=DIRECTION ( 'NONE',  ( -0.000000000000000000, 1.000000000000000000, -0.000000000000000000 ) ) ;
#101859=ORIENTED_EDGE ( 'NONE', *, *, #20516, .F. ) ;
#101860=EDGE_CURVE ( 'NONE', #48260, #66886, #102516, .T. ) ;
#101861=ADVANCED_FACE ( 'NONE', ( #64978 ), #52340, .T. ) ;
#101862=EDGE_CURVE ( 'NONE', #94029, #13624, #84637, .T. ) ;
#101863=EDGE_CURVE ( 'NONE', #108453, #251, #104901, .T. ) ;
#101864=EDGE_CURVE ( 'NONE', #99586, #70146, #104278, .T. ) ;
#101865=CIRCLE ( 'NONE', #89251, 0.1000000000000000056 ) ;
#101866=ORIENTED_EDGE ( 'NONE', *, *, #112203, .F. ) ;
#101867=AXIS2_PLACEMENT_3D ( 'NONE', #15141, #125127, #15799 ) ;
#101868=DIRECTION ( 'NONE',  ( 0.000000000000000000, -0.9999939076577903929, 0.003490651415223739937 ) ) ;
#101869=ORIENTED_EDGE ( 'NONE', *, *, #33586, .F. ) ;
#101870=ORIENTED_EDGE ( 'NONE', *, *, #14381, .F. ) ;
#101871=CARTESIAN_POINT ( 'NONE',  ( 6.249999999999930722, 2.500000000000000000, -1.572243186433550211 ) ) ;
#101872=EDGE_CURVE ( 'NONE', #125678, #21143, #74818, .T. ) ;
#101873=VECTOR ( 'NONE', #79555, 1000.000000000000000 ) ;
#101874=DIRECTION ( 'NONE',  ( 0.000000000000000000, 0.000000000000000000, 1.000000000000000000 ) ) ;
#101875=CARTESIAN_POINT ( 'NONE',  ( -2.100000000000033840, 12.50000000000000000, 3.637306695894644726 ) ) ;
#101876=CIRCLE ( 'NONE', #37039, 0.06509327318403741736 ) ;
#101877=DIRECTION ( 'NONE',  ( -0.000000000000000000, -1.000000000000000000, -0.000000000000000000 ) ) ;
#101878=EDGE_LOOP ( 'NONE', ( #13855, #122561 ) ) ;
#101879=AXIS2_PLACEMENT_3D ( 'NONE', #64149, #73980, #66081 ) ;
#101880=AXIS2_PLACEMENT_3D ( 'NONE', #128942, #71275, #119097 ) ;
#101881=FACE_OUTER_BOUND ( 'NONE', #89248, .T. ) ;
#101882=ORIENTED_EDGE ( 'NONE', *, *, #60312, .F. ) ;
#101883=CARTESIAN_POINT ( 'NONE',  ( 17.50000000000000000, 2.500000000000000000, 2.922290670087886344 ) ) ;
#101884=AXIS2_PLACEMENT_3D ( 'NONE', #121585, #52222, #113056 ) ;
#101885=LINE ( 'NONE', #92051, #73952 ) ;
#101887=CONICAL_SURFACE ( 'NONE', #118605, 0.09999999999999982514, 0.003490658503988666988 ) ;
#101888=AXIS2_PLACEMENT_3D ( 'NONE', #63294, #111757, #103228 ) ;
#101889=ORIENTED_EDGE ( 'NONE', *, *, #93318, .T. ) ;
#101890=ORIENTED_EDGE ( 'NONE', *, *, #35881, .F. ) ;
#101891=VERTEX_POINT ( 'NONE', #125207 ) ;
#101892=DIRECTION ( 'NONE',  ( 0.000000000000000000, 0.000000000000000000, 1.000000000000000000 ) ) ;
#101893=CARTESIAN_POINT ( 'NONE',  ( 13.91976764310571824, 2.500000000000000444, 6.779443705067744297 ) ) ;
#101894=PLANE ( 'NONE',  #62954 ) ;
#101895=FACE_BOUND ( 'NONE', #41609, .T. ) ;
#101896=ORIENTED_EDGE ( 'NONE', *, *, #107699, .F. ) ;
#101897=PLANE ( 'NONE',  #97494 ) ;
#101899=DIRECTION ( 'NONE',  ( 0.000000000000000000, 0.000000000000000000, -1.000000000000000000 ) ) ;
#101900=CARTESIAN_POINT ( 'NONE',  ( -11.64999999999999680, 2.500000000000000000, 6.595190528383296780 ) ) ;
#101901=DIRECTION ( 'NONE',  ( 0.000000000000000000, -0.000000000000000000, 1.000000000000000000 ) ) ;
#101903=EDGE_CURVE ( 'NONE', #62359, #44343, #112168, .T. ) ;
#101905=CARTESIAN_POINT ( 'NONE',  ( -6.249999999999984901, 2.500000000000000000, -2.265063509461101798 ) ) ;
#101906=EDGE_CURVE ( 'NONE', #2854, #87563, #12654, .T. ) ;
#101907=DIRECTION ( 'NONE',  ( 0.000000000000000000, 0.000000000000000000, -1.000000000000000000 ) ) ;
#101908=EDGE_CURVE ( 'NONE', #128585, #72457, #94113, .T. ) ;
#101909=EDGE_LOOP ( 'NONE', ( #116736, #28863 ) ) ;
#101910=ORIENTED_EDGE ( 'NONE', *, *, #2530, .T. ) ;
#101911=ORIENTED_EDGE ( 'NONE', *, *, #51906, .F. ) ;
#101912=ORIENTED_EDGE ( 'NONE', *, *, #95178, .F. ) ;
#101913=VERTEX_POINT ( 'NONE', #2850 ) ;
#101914=DIRECTION ( 'NONE',  ( 0.000000000000000000, 1.000000000000000000, 0.000000000000000000 ) ) ;
#101915=DIRECTION ( 'NONE',  ( 0.000000000000000000, 1.000000000000000000, 0.000000000000000000 ) ) ;
#101916=ORIENTED_EDGE ( 'NONE', *, *, #50966, .F. ) ;
#101917=EDGE_CURVE ( 'NONE', #3186, #78294, #110827, .T. ) ;
#101918=FACE_BOUND ( 'NONE', #23074, .T. ) ;
#101919=DIRECTION ( 'NONE',  ( -0.000000000000000000, -1.000000000000000000, -0.000000000000000000 ) ) ;
#101920=EDGE_CURVE ( 'NONE', #13968, #125307, #114733, .T. ) ;
#101921=CIRCLE ( 'NONE', #5745, 0.06509327318403745899 ) ;
#101922=ADVANCED_FACE ( 'NONE', ( #13950 ), #54515, .T. ) ;
#101923=CIRCLE ( 'NONE', #43354, 0.06509327318403745899 ) ;
#101924=ADVANCED_FACE ( 'NONE', ( #123907 ), #113068, .T. ) ;
#101925=ORIENTED_EDGE ( 'NONE', *, *, #41174, .T. ) ;
#101926=CARTESIAN_POINT ( 'NONE',  ( 3.749999999999942268, 12.50000000000000000, 1.472243186433545459 ) ) ;
#101927=CARTESIAN_POINT ( 'NONE',  ( 6.249999999999932498, 2.500000000000000000, 5.802370205355744659 ) ) ;
#101928=CARTESIAN_POINT ( 'NONE',  ( -7.300000000000013145, 2.500000000000000000, 3.983716857408420076 ) ) ;
#101929=ORIENTED_EDGE ( 'NONE', *, *, #86853, .T. ) ;
#101930=CARTESIAN_POINT ( 'NONE',  ( -2.499999999999996003, 12.50000000000000000, -4.265033745738164406 ) ) ;
#101931=EDGE_CURVE ( 'NONE', #1738, #43544, #44723, .T. ) ;
#101932=CIRCLE ( 'NONE', #43364, 0.06509327318403745899 ) ;
#101933=EDGE_LOOP ( 'NONE', ( #89510, #67569 ) ) ;
#101934=VERTEX_POINT ( 'NONE', #36837 ) ;
#101935=ORIENTED_EDGE ( 'NONE', *, *, #107985, .F. ) ;
#101937=DIRECTION ( 'NONE',  ( 0.000000000000000000, -0.9999939076577903929, 0.003490651415223739937 ) ) ;
#101938=ORIENTED_EDGE ( 'NONE', *, *, #11314, .F. ) ;
#101939=LINE ( 'NONE', #72487, #72652 ) ;
#101940=CIRCLE ( 'NONE', #87340, 0.09999999999999982514 ) ;
#101941=FACE_OUTER_BOUND ( 'NONE', #92764, .T. ) ;
#101942=DIRECTION ( 'NONE',  ( 0.000000000000000000, 1.000000000000000000, 0.000000000000000000 ) ) ;
#101943=DIRECTION ( 'NONE',  ( 0.000000000000000000, 0.000000000000000000, 1.000000000000000000 ) ) ;
#101944=ORIENTED_EDGE ( 'NONE', *, *, #43053, .F. ) ;
#101945=DIRECTION ( 'NONE',  ( 0.000000000000000000, -0.000000000000000000, 1.000000000000000000 ) ) ;
#101946=EDGE_CURVE ( 'NONE', #125134, #125433, #50379, .T. ) ;
#101947=EDGE_LOOP ( 'NONE', ( #10829, #58519, #112610, #19799 ) ) ;
#101948=DIRECTION ( 'NONE',  ( 0.000000000000000000, 0.000000000000000000, 1.000000000000000000 ) ) ;
#101949=VERTEX_POINT ( 'NONE', #117280 ) ;
#101950=FACE_OUTER_BOUND ( 'NONE', #54909, .T. ) ;
#101951=ORIENTED_EDGE ( 'NONE', *, *, #123783, .T. ) ;
#101952=LINE ( 'NONE', #120939, #72221 ) ;
#101953=AXIS2_PLACEMENT_3D ( 'NONE', #106752, #107408, #8540 ) ;
#101954=DIRECTION ( 'NONE',  ( 0.000000000000000000, 1.000000000000000000, 0.000000000000000000 ) ) ;
#101955=DIRECTION ( 'NONE',  ( 0.000000000000000000, 1.000000000000000000, 0.000000000000000000 ) ) ;
#101956=LINE ( 'NONE', #72506, #65502 ) ;
#101957=CARTESIAN_POINT ( 'NONE',  ( 3.549999999999944755, 12.50000000000000000, -6.841600689897077814 ) ) ;
#101958=CIRCLE ( 'NONE', #106065, 0.1000000000000000472 ) ;
#101959=ORIENTED_EDGE ( 'NONE', *, *, #20211, .T. ) ;
#101960=VECTOR ( 'NONE', #101468, 1000.000000000000000 ) ;
#101961=ORIENTED_EDGE ( 'NONE', *, *, #75564, .T. ) ;
#101962=PLANE ( 'NONE',  #22491 ) ;
#101963=AXIS2_PLACEMENT_3D ( 'NONE', #98311, #6686, #46655 ) ;
#101964=EDGE_CURVE ( 'NONE', #16412, #14739, #48585, .T. ) ;
#101965=CARTESIAN_POINT ( 'NONE',  ( 12.69999999999990159, 2.500000000000000000, -3.883716857408426648 ) ) ;
#101966=DIRECTION ( 'NONE',  ( -0.000000000000000000, -1.000000000000000000, -0.000000000000000000 ) ) ;
#101967=ORIENTED_EDGE ( 'NONE', *, *, #14488, .F. ) ;
#101968=EDGE_LOOP ( 'NONE', ( #97239, #9556, #53018, #114594 ) ) ;
#101969=EDGE_LOOP ( 'NONE', ( #75209, #69159 ) ) ;
#101970=DIRECTION ( 'NONE',  ( 0.000000000000000000, 0.000000000000000000, 1.000000000000000000 ) ) ;
#101971=AXIS2_PLACEMENT_3D ( 'NONE', #98374, #50572, #61040 ) ;
#101972=AXIS2_PLACEMENT_3D ( 'NONE', #56526, #74895, #114174 ) ;
#101973=VERTEX_POINT ( 'NONE', #107500 ) ;
#101974=DIRECTION ( 'NONE',  ( 0.000000000000000000, 0.000000000000000000, 1.000000000000000000 ) ) ;
#101975=DIRECTION ( 'NONE',  ( 0.000000000000000000, 0.000000000000000000, 1.000000000000000000 ) ) ;
#101976=AXIS2_PLACEMENT_3D ( 'NONE', #114421, #92873, #103330 ) ;
#101977=DIRECTION ( 'NONE',  ( -4.274815082592931898E-19, -0.9999939076577903929, -0.003490651415223739937 ) ) ;
#101978=ORIENTED_EDGE ( 'NONE', *, *, #13180, .T. ) ;
#101979=CARTESIAN_POINT ( 'NONE',  ( -9.800000000000006040, 12.50000000000000000, 0.3464101615137735735 ) ) ;
#101980=DIRECTION ( 'NONE',  ( 0.000000000000000000, 1.000000000000000000, 0.000000000000000000 ) ) ;
#101981=DIRECTION ( 'NONE',  ( -4.274815082592931898E-19, -0.9999939076577903929, -0.003490651415223739937 ) ) ;
#101982=CARTESIAN_POINT ( 'NONE',  ( -10.00000000000000355, 12.50000000000000000, 3.637306695894644726 ) ) ;
#101983=AXIS2_PLACEMENT_3D ( 'NONE', #1176, #70559, #110486 ) ;
#101984=EDGE_CURVE ( 'NONE', #27644, #109941, #7996, .T. ) ;
#101985=CARTESIAN_POINT ( 'NONE',  ( 7.899999999999923084, 12.50000000000000000, -0.6928203230275542523 ) ) ;
#101986=ORIENTED_EDGE ( 'NONE', *, *, #102325, .T. ) ;
#101987=FACE_OUTER_BOUND ( 'NONE', #25488, .T. ) ;
#101988=AXIS2_PLACEMENT_3D ( 'NONE', #43396, #11341, #83316 ) ;
#101989=AXIS2_PLACEMENT_3D ( 'NONE', #59955, #18051, #29823 ) ;
#101990=CARTESIAN_POINT ( 'NONE',  ( 59.88499455099038471, -2.860410828927322680, 5.641292085222127106 ) ) ;
#101991=ORIENTED_EDGE ( 'NONE', *, *, #17150, .T. ) ;
#101992=ORIENTED_EDGE ( 'NONE', *, *, #10873, .T. ) ;
#101994=DIRECTION ( 'NONE',  ( -4.274815082592931898E-19, -0.9999939076577903929, -0.003490651415223739937 ) ) ;
#101996=DIRECTION ( 'NONE',  ( 0.000000000000000000, 0.000000000000000000, 1.000000000000000000 ) ) ;
#101997=DIRECTION ( 'NONE',  ( 0.000000000000000000, 0.000000000000000000, -1.000000000000000000 ) ) ;
#101998=DIRECTION ( 'NONE',  ( 0.000000000000000000, 0.000000000000000000, -1.000000000000000000 ) ) ;
#101999=FACE_OUTER_BOUND ( 'NONE', #51507, .T. ) ;
#102000=CARTESIAN_POINT ( 'NONE',  ( -2.300000000000033129, 2.500000000000000000, 3.983716857408420076 ) ) ;
#102001=LINE ( 'NONE', #120993, #58381 ) ;
#102002=EDGE_LOOP ( 'NONE', ( #104001, #26411 ) ) ;
#102003=ORIENTED_EDGE ( 'NONE', *, *, #90837, .F. ) ;
#102004=ADVANCED_FACE ( 'NONE', ( #106835 ), #108136, .T. ) ;
#102005=ORIENTED_EDGE ( 'NONE', *, *, #80856, .F. ) ;
#102006=AXIS2_PLACEMENT_3D ( 'NONE', #79712, #20153, #60094 ) ;
#102007=ORIENTED_EDGE ( 'NONE', *, *, #20560, .F. ) ;
#102008=LINE ( 'NONE', #12328, #12737 ) ;
#102009=DIRECTION ( 'NONE',  ( -0.000000000000000000, 1.000000000000000000, -0.000000000000000000 ) ) ;
#102010=EDGE_LOOP ( 'NONE', ( #90985, #121314 ) ) ;
#102011=CIRCLE ( 'NONE', #129230, 0.1000000000000002554 ) ;
#102012=CARTESIAN_POINT ( 'NONE',  ( 11.24999999999991118, 12.50000000000000000, 5.737276932171707422 ) ) ;
#102013=CIRCLE ( 'NONE', #58105, 0.06509327318403745899 ) ;
#102014=DIRECTION ( 'NONE',  ( -0.000000000000000000, -1.000000000000000000, -0.000000000000000000 ) ) ;
#102015=DIRECTION ( 'NONE',  ( 0.000000000000000000, -0.9999939076577903929, 0.003490651415223739937 ) ) ;
#102016=ORIENTED_EDGE ( 'NONE', *, *, #105638, .T. ) ;
#102017=ADVANCED_FACE ( 'NONE', ( #116666 ), #97033, .T. ) ;
#102018=EDGE_CURVE ( 'NONE', #44623, #37437, #66998, .T. ) ;
#102019=EDGE_CURVE ( 'NONE', #83059, #51134, #27291, .T. ) ;
#102020=CARTESIAN_POINT ( 'NONE',  ( 9.149999999999918643, 12.50000000000000000, 2.230156782645134950 ) ) ;
#102021=ADVANCED_FACE ( 'NONE', ( #77395 ), #46172, .T. ) ;
#102022=AXIS2_PLACEMENT_3D ( 'NONE', #49360, #29698, #81839 ) ;
#102023=DIRECTION ( 'NONE',  ( -0.000000000000000000, 1.000000000000000000, -0.000000000000000000 ) ) ;
#102024=EDGE_LOOP ( 'NONE', ( #12582, #123764, #111707, #86596 ) ) ;
#102025=AXIS2_PLACEMENT_3D ( 'NONE', #91580, #81747, #41215 ) ;
#102026=ORIENTED_EDGE ( 'NONE', *, *, #119197, .F. ) ;
#102027=ORIENTED_EDGE ( 'NONE', *, *, #50038, .F. ) ;
#102028=VERTEX_POINT ( 'NONE', #26371 ) ;
#102029=FACE_OUTER_BOUND ( 'NONE', #74590, .T. ) ;
#102030=ADVANCED_FACE ( 'NONE', ( #105568 ), #12704, .T. ) ;
#102031=DIRECTION ( 'NONE',  ( -0.000000000000000000, -1.000000000000000000, -0.000000000000000000 ) ) ;
#102032=CARTESIAN_POINT ( 'NONE',  ( -11.24999999999996447, 12.50000000000000000, -6.495190528383298911 ) ) ;
#102033=EDGE_CURVE ( 'NONE', #108138, #106136, #50297, .T. ) ;
#102034=CARTESIAN_POINT ( 'NONE',  ( -6.850000000000017408, 12.50000000000000000, -1.753560074763288457 ) ) ;
#102035=CIRCLE ( 'NONE', #64367, 0.06509327318403745899 ) ;
#102036=ADVANCED_FACE ( 'NONE', ( #47943 ), #83740, .T. ) ;
#102037=ORIENTED_EDGE ( 'NONE', *, *, #112640, .T. ) ;
#102038=DIRECTION ( 'NONE',  ( 0.000000000000000000, 1.000000000000000000, 0.000000000000000000 ) ) ;
#102041=DIRECTION ( 'NONE',  ( 0.000000000000000000, 0.000000000000000000, -1.000000000000000000 ) ) ;
#102042=DIRECTION ( 'NONE',  ( 0.000000000000000000, 0.000000000000000000, 1.000000000000000000 ) ) ;
#102043=DIRECTION ( 'NONE',  ( -0.000000000000000000, -1.000000000000000000, -0.000000000000000000 ) ) ;
#102044=ORIENTED_EDGE ( 'NONE', *, *, #13973, .F. ) ;
#102045=AXIS2_PLACEMENT_3D ( 'NONE', #40737, #10581, #51829 ) ;
#102046=CONICAL_SURFACE ( 'NONE', #53922, 0.09999999999999982514, 0.003490658503988666988 ) ;
#102047=VERTEX_POINT ( 'NONE', #98307 ) ;
#102048=ORIENTED_EDGE ( 'NONE', *, *, #106127, .T. ) ;
#102049=CARTESIAN_POINT ( 'NONE',  ( -9.150000000000009237, 2.500000000000000000, -1.572243186433550211 ) ) ;
#102050=CARTESIAN_POINT ( 'NONE',  ( -6.450000000000016165, 2.500000000000000000, 6.941600689897073018 ) ) ;
#102051=DIRECTION ( 'NONE',  ( 0.000000000000000000, 0.000000000000000000, -1.000000000000000000 ) ) ;
#102052=FACE_BOUND ( 'NONE', #4638, .T. ) ;
#102053=VECTOR ( 'NONE', #7443, 1000.000000000000000 ) ;
#102054=CARTESIAN_POINT ( 'NONE',  ( -2.500000000000032863, 12.50000000000000000, 4.957854068765711553 ) ) ;
#102055=CARTESIAN_POINT ( 'NONE',  ( -6.249999999999981348, 2.500000000000000000, 2.165063509461097713 ) ) ;
#102056=CIRCLE ( 'NONE', #14202, 0.09999999999999982514 ) ;
#102057=CARTESIAN_POINT ( 'NONE',  ( -4.999999999999986677, 12.50000000000000000, -2.276824562219559311E-15 ) ) ;
#102058=AXIS2_PLACEMENT_3D ( 'NONE', #11864, #40719, #89793 ) ;
#102060=DIRECTION ( 'NONE',  ( 0.000000000000000000, 1.000000000000000000, 0.000000000000000000 ) ) ;
#102061=CIRCLE ( 'NONE', #45638, 0.06509327318403745899 ) ;
#102063=LINE ( 'NONE', #2543, #7212 ) ;
#102064=EDGE_LOOP ( 'NONE', ( #35949, #65366, #54883, #61830 ) ) ;
#102065=DIRECTION ( 'NONE',  ( 0.000000000000000000, 0.000000000000000000, -1.000000000000000000 ) ) ;
#102066=DIRECTION ( 'NONE',  ( 0.000000000000000000, 0.000000000000000000, 1.000000000000000000 ) ) ;
#102068=VERTEX_POINT ( 'NONE', #70792 ) ;
#102069=CARTESIAN_POINT ( 'NONE',  ( -7.050000000000016698, 2.500000000000000000, -6.495190528383302464 ) ) ;
#102070=CONICAL_SURFACE ( 'NONE', #26847, 0.09999999999999982514, 0.003490658503988666988 ) ;
#102071=CARTESIAN_POINT ( 'NONE',  ( -14.59999999999998366, 2.500000000000000000, -0.1000000000000001166 ) ) ;
#102072=FACE_BOUND ( 'NONE', #25950, .T. ) ;
#102073=DIRECTION ( 'NONE',  ( 0.000000000000000000, -0.000000000000000000, 1.000000000000000000 ) ) ;
#102074=EDGE_CURVE ( 'NONE', #67061, #73868, #29460, .T. ) ;
#102075=AXIS2_PLACEMENT_3D ( 'NONE', #103279, #103917, #32633 ) ;
#102076=CIRCLE ( 'NONE', #62379, 0.1000000000000002554 ) ;
#102077=ADVANCED_FACE ( 'NONE', ( #99622 ), #51170, .T. ) ;
#102078=ORIENTED_EDGE ( 'NONE', *, *, #42693, .F. ) ;
#102079=FACE_OUTER_BOUND ( 'NONE', #72626, .T. ) ;
#102080=DIRECTION ( 'NONE',  ( 0.000000000000000000, 1.000000000000000000, 0.000000000000000000 ) ) ;
#102081=EDGE_LOOP ( 'NONE', ( #119660, #56476 ) ) ;
#102082=CARTESIAN_POINT ( 'NONE',  ( 0.3999999999999568345, 12.50000000000000000, -3.637306695894650055 ) ) ;
#102083=CARTESIAN_POINT ( 'NONE',  ( -11.64999999999999680, 12.50000000000000000, 1.472243186433545459 ) ) ;
#102085=ORIENTED_EDGE ( 'NONE', *, *, #55766, .T. ) ;
#102086=AXIS2_PLACEMENT_3D ( 'NONE', #124936, #113173, #23504 ) ;
#102087=DIRECTION ( 'NONE',  ( -0.000000000000000000, 1.000000000000000000, -0.000000000000000000 ) ) ;
#102088=DIRECTION ( 'NONE',  ( 0.000000000000000000, 1.000000000000000000, 0.000000000000000000 ) ) ;
#102089=VERTEX_POINT ( 'NONE', #128452 ) ;
#102090=CARTESIAN_POINT ( 'NONE',  ( 10.19999999999991225, 12.50000000000000000, -4.611443907251940644 ) ) ;
#102091=CIRCLE ( 'NONE', #66858, 0.1000000000000002554 ) ;
#102092=CARTESIAN_POINT ( 'NONE',  ( 11.24999999999990763, 2.500000000000000000, -7.188010851410854052 ) ) ;
#102093=CIRCLE ( 'NONE', #93682, 0.09999999999999982514 ) ;
#102094=CONICAL_SURFACE ( 'NONE', #77242, 0.1000000000000002554, 0.003490658503988666988 ) ;
#102095=DIRECTION ( 'NONE',  ( -4.274815082592931898E-19, -0.9999939076577903929, -0.003490651415223739937 ) ) ;
#102096=EDGE_LOOP ( 'NONE', ( #7985, #57549, #78252, #6076 ) ) ;
#102097=ORIENTED_EDGE ( 'NONE', *, *, #95925, .F. ) ;
#102098=CARTESIAN_POINT ( 'NONE',  ( -3.300000000000028244, 12.50000000000000000, 4.330127018922196314 ) ) ;
#102099=CIRCLE ( 'NONE', #8094, 0.1000000000000002554 ) ;
#102101=CARTESIAN_POINT ( 'NONE',  ( -14.79999999999998472, 12.50000000000000000, 0.3464101615137758494 ) ) ;
#102102=CARTESIAN_POINT ( 'NONE',  ( -4.350000000000023626, 2.500000000000000000, 6.148780366869520897 ) ) ;
#102103=VECTOR ( 'NONE', #65418, 1000.000000000000000 ) ;
#102104=CIRCLE ( 'NONE', #110408, 0.1000000000000002554 ) ;
#102105=CARTESIAN_POINT ( 'NONE',  ( -3.300000000000027800, 2.500000000000000000, -2.276824562219559311E-15 ) ) ;
#102106=ORIENTED_EDGE ( 'NONE', *, *, #17478, .F. ) ;
#102107=FACE_OUTER_BOUND ( 'NONE', #67329, .T. ) ;
#102108=LINE ( 'NONE', #99540, #7989 ) ;
#102109=CARTESIAN_POINT ( 'NONE',  ( 4.399999999999939071, 2.500000000000000000, 0.3464101615137736845 ) ) ;
#102110=CARTESIAN_POINT ( 'NONE',  ( 7.949999999999925571, 12.50000000000000000, 2.099970236277060032 ) ) ;
#102111=DIRECTION ( 'NONE',  ( 0.000000000000000000, 1.000000000000000000, 0.000000000000000000 ) ) ;
#102112=CARTESIAN_POINT ( 'NONE',  ( -9.400000000000007461, 2.500000000000000000, -0.2464101615137783419 ) ) ;
#102113=AXIS2_PLACEMENT_3D ( 'NONE', #99320, #9642, #88172 ) ;
#102114=EDGE_LOOP ( 'NONE', ( #71467, #101446, #82316, #111489 ) ) ;
#102115=CIRCLE ( 'NONE', #89597, 0.1000000000000000056 ) ;
#102116=VERTEX_POINT ( 'NONE', #110079 ) ;
#102117=CARTESIAN_POINT ( 'NONE',  ( 9.999999999999916511, 12.50000000000000000, -0.6277270498435166823 ) ) ;
#102118=ORIENTED_EDGE ( 'NONE', *, *, #126855, .F. ) ;
#102119=ADVANCED_FACE ( 'NONE', ( #10566 ), #127650, .T. ) ;
#102121=VERTEX_POINT ( 'NONE', #110707 ) ;
#102122=ORIENTED_EDGE ( 'NONE', *, *, #106463, .F. ) ;
#102123=VERTEX_POINT ( 'NONE', #31517 ) ;
#102124=CARTESIAN_POINT ( 'NONE',  ( 9.199999999999915801, 2.500000000000000000, -4.230127018922201998 ) ) ;
#102125=CARTESIAN_POINT ( 'NONE',  ( 11.44999999999991047, 12.50000000000000000, 6.148780366869520009 ) ) ;
#102126=DIRECTION ( 'NONE',  ( 0.000000000000000000, 0.000000000000000000, 1.000000000000000000 ) ) ;
#102128=PLANE ( 'NONE',  #43190 ) ;
#102129=CARTESIAN_POINT ( 'NONE',  ( -11.84999999999999787, 2.500000000000000000, -2.511473670974873951 ) ) ;
#102130=CIRCLE ( 'NONE', #118844, 0.06509327318403745899 ) ;
#102131=CARTESIAN_POINT ( 'NONE',  ( -2.100000000000033396, 2.500000000000000000, -5.022947341949754119 ) ) ;
#102132=ADVANCED_FACE ( 'NONE', ( #758 ), #62904, .T. ) ;
#102133=FACE_OUTER_BOUND ( 'NONE', #57863, .T. ) ;
#102134=CIRCLE ( 'NONE', #79064, 0.09999999999999999167 ) ;
#102135=DIRECTION ( 'NONE',  ( 0.000000000000000000, 0.000000000000000000, 1.000000000000000000 ) ) ;
#102136=EDGE_CURVE ( 'NONE', #18789, #119556, #119330, .T. ) ;
#102137=PLANE ( 'NONE',  #66585 ) ;
#102138=AXIS2_PLACEMENT_3D ( 'NONE', #69294, #7805, #17622 ) ;
#102139=ORIENTED_EDGE ( 'NONE', *, *, #25916, .F. ) ;
#102141=PLANE ( 'NONE',  #23511 ) ;
#102142=ORIENTED_EDGE ( 'NONE', *, *, #7231, .T. ) ;
#102143=EDGE_CURVE ( 'NONE', #35473, #8018, #6425, .T. ) ;
#102144=ORIENTED_EDGE ( 'NONE', *, *, #25911, .F. ) ;
#102145=CARTESIAN_POINT ( 'NONE',  ( 6.449999999999931788, 2.500000000000000000, -2.611473670974877592 ) ) ;
#102146=DIRECTION ( 'NONE',  ( 0.000000000000000000, 0.000000000000000000, 1.000000000000000000 ) ) ;
#102147=AXIS2_PLACEMENT_3D ( 'NONE', #13412, #63165, #15336 ) ;
#102148=DIRECTION ( 'NONE',  ( -0.000000000000000000, -1.000000000000000000, -0.000000000000000000 ) ) ;
#102149=CARTESIAN_POINT ( 'NONE',  ( 4.399999999999940847, 12.50000000000000000, -3.983716857408426293 ) ) ;
#102150=LINE ( 'NONE', #9899, #8774 ) ;
#102151=DIRECTION ( 'NONE',  ( -0.000000000000000000, -1.000000000000000000, -0.000000000000000000 ) ) ;
#102152=DIRECTION ( 'NONE',  ( -4.274815082592931898E-19, -0.9999939076577903929, -0.003490651415223739937 ) ) ;
#102153=ORIENTED_EDGE ( 'NONE', *, *, #41618, .F. ) ;
#102154=CIRCLE ( 'NONE', #20584, 0.09999999999999982514 ) ;
#102156=VERTEX_POINT ( 'NONE', #21044 ) ;
#102157=EDGE_CURVE ( 'NONE', #69509, #81044, #90073, .T. ) ;
#102158=CIRCLE ( 'NONE', #96167, 0.06509327318403745899 ) ;
#102160=CONICAL_SURFACE ( 'NONE', #100108, 0.1000000000000002554, 0.003490658503988666988 ) ;
#102161=VERTEX_POINT ( 'NONE', #9941 ) ;
#102162=DIRECTION ( 'NONE',  ( 0.000000000000000000, 1.000000000000000000, 0.000000000000000000 ) ) ;
#102163=LINE ( 'NONE', #12483, #83349 ) ;
#102164=EDGE_CURVE ( 'NONE', #249, #25677, #37772, .T. ) ;
#102165=CONICAL_SURFACE ( 'NONE', #120934, 0.1000000000000002554, 0.003490658503988666988 ) ;
#102166=CIRCLE ( 'NONE', #54046, 0.1000000000000002554 ) ;
#102167=CARTESIAN_POINT ( 'NONE',  ( -12.29999999999999361, 12.50000000000000000, 3.983716857408420076 ) ) ;
#102168=DIRECTION ( 'NONE',  ( 0.000000000000000000, -0.9999939076577903929, 0.003490651415223739937 ) ) ;
#102169=CARTESIAN_POINT ( 'NONE',  ( -8.950000000000008171, 2.500000000000000000, -2.611473670974877592 ) ) ;
#102170=VERTEX_POINT ( 'NONE', #11861 ) ;
#102171=CARTESIAN_POINT ( 'NONE',  ( 1.449999999999951328, 12.50000000000000000, 2.511473670974873507 ) ) ;
#102172=CARTESIAN_POINT ( 'NONE',  ( 1.449999999999950440, 2.500000000000000000, 6.148780366869520009 ) ) ;
#102173=EDGE_CURVE ( 'NONE', #28294, #1556, #25227, .T. ) ;
#102174=EDGE_CURVE ( 'NONE', #126006, #43603, #9297, .T. ) ;
#102175=CARTESIAN_POINT ( 'NONE',  ( -1.250000000000037970, 2.500000000000000000, 2.957883832488649389 ) ) ;
#102176=EDGE_CURVE ( 'NONE', #95189, #67065, #49886, .T. ) ;
#102177=DIRECTION ( 'NONE',  ( 0.000000000000000000, 1.000000000000000000, 0.000000000000000000 ) ) ;
#102178=EDGE_CURVE ( 'NONE', #27833, #105130, #123528, .T. ) ;
#102179=DIRECTION ( 'NONE',  ( -0.000000000000000000, -1.000000000000000000, -0.000000000000000000 ) ) ;
#102180=ORIENTED_EDGE ( 'NONE', *, *, #124846, .T. ) ;
#102181=EDGE_LOOP ( 'NONE', ( #103919, #71795, #113500, #117915 ) ) ;
#102182=EDGE_CURVE ( 'NONE', #91287, #115300, #121384, .T. ) ;
#102183=ORIENTED_EDGE ( 'NONE', *, *, #98326, .F. ) ;
#102184=LINE ( 'NONE', #90405, #6993 ) ;
#102185=ADVANCED_FACE ( 'NONE', ( #21705 ), #129102, .T. ) ;
#102186=VERTEX_POINT ( 'NONE', #40052 ) ;
#102187=DIRECTION ( 'NONE',  ( 0.000000000000000000, 0.000000000000000000, 1.000000000000000000 ) ) ;
#102188=DIRECTION ( 'NONE',  ( 0.000000000000000000, 0.000000000000000000, 1.000000000000000000 ) ) ;
#102189=EDGE_CURVE ( 'NONE', #124289, #44948, #101547, .T. ) ;
#102190=CIRCLE ( 'NONE', #16565, 0.1000000000000002554 ) ;
#102191=EDGE_CURVE ( 'NONE', #115959, #41978, #58701, .T. ) ;
#102192=AXIS2_PLACEMENT_3D ( 'NONE', #48070, #97160, #7479 ) ;
#102193=AXIS2_PLACEMENT_3D ( 'NONE', #79746, #119663, #69931 ) ;
#102194=ORIENTED_EDGE ( 'NONE', *, *, #82364, .F. ) ;
#102195=DIRECTION ( 'NONE',  ( 0.000000000000000000, -0.9999939076577903929, 0.003490651415223739937 ) ) ;
#102196=DIRECTION ( 'NONE',  ( -0.000000000000000000, -1.000000000000000000, -0.000000000000000000 ) ) ;
#102197=EDGE_CURVE ( 'NONE', #83000, #42689, #25324, .T. ) ;
#102198=DIRECTION ( 'NONE',  ( -0.000000000000000000, 1.000000000000000000, -0.000000000000000000 ) ) ;
#102199=DIRECTION ( 'NONE',  ( 0.000000000000000000, -0.9999939076577903929, 0.003490651415223739937 ) ) ;
#102200=EDGE_CURVE ( 'NONE', #13735, #109941, #54564, .T. ) ;
#102201=AXIS2_PLACEMENT_3D ( 'NONE', #127920, #55952, #6195 ) ;
#102202=AXIS2_PLACEMENT_3D ( 'NONE', #91512, #100668, #60145 ) ;
#102203=CONICAL_SURFACE ( 'NONE', #114705, 0.09999999999999982514, 0.003490658503988666988 ) ;
#102204=DIRECTION ( 'NONE',  ( -0.000000000000000000, 1.000000000000000000, -0.000000000000000000 ) ) ;
#102206=EDGE_LOOP ( 'NONE', ( #26840, #82051 ) ) ;
#102207=LINE ( 'NONE', #23000, #39732 ) ;
#102208=CARTESIAN_POINT ( 'NONE',  ( -9.350000000000006750, 2.500000000000000000, 2.411473670974873862 ) ) ;
#102209=LINE ( 'NONE', #12517, #30434 ) ;
#102210=DIRECTION ( 'NONE',  ( 0.000000000000000000, 0.000000000000000000, -1.000000000000000000 ) ) ;
#102211=AXIS2_PLACEMENT_3D ( 'NONE', #43118, #103304, #13611 ) ;
#102212=ORIENTED_EDGE ( 'NONE', *, *, #40226, .F. ) ;
#102213=VERTEX_POINT ( 'NONE', #104740 ) ;
#102214=DIRECTION ( 'NONE',  ( 0.000000000000000000, 0.000000000000000000, -1.000000000000000000 ) ) ;
#102215=DIRECTION ( 'NONE',  ( 0.000000000000000000, 0.000000000000000000, 1.000000000000000000 ) ) ;
#102216=CARTESIAN_POINT ( 'NONE',  ( 6.449999999999930012, 2.500000000000000000, 6.741600689897071952 ) ) ;
#102217=DIRECTION ( 'NONE',  ( 0.000000000000000000, 0.000000000000000000, -1.000000000000000000 ) ) ;
#102218=ORIENTED_EDGE ( 'NONE', *, *, #49773, .T. ) ;
#102219=CONICAL_SURFACE ( 'NONE', #118934, 0.1000000000000002554, 0.003490658503988666988 ) ;
#102220=DIRECTION ( 'NONE',  ( 0.000000000000000000, 1.000000000000000000, 0.000000000000000000 ) ) ;
#102221=DIRECTION ( 'NONE',  ( 0.000000000000000000, 0.000000000000000000, 1.000000000000000000 ) ) ;
#102222=AXIS2_PLACEMENT_3D ( 'NONE', #41335, #111315, #124227 ) ;
#102223=VERTEX_POINT ( 'NONE', #24268 ) ;
#102224=DIRECTION ( 'NONE',  ( 0.000000000000000000, -0.000000000000000000, 1.000000000000000000 ) ) ;
#102225=ORIENTED_EDGE ( 'NONE', *, *, #114548, .F. ) ;
#102226=CARTESIAN_POINT ( 'NONE',  ( 11.69999999999990870, 2.500000000000000000, -4.330127018922201643 ) ) ;
#102228=ORIENTED_EDGE ( 'NONE', *, *, #85250, .F. ) ;
#102229=AXIS2_PLACEMENT_3D ( 'NONE', #120828, #22005, #51460 ) ;
#102230=CARTESIAN_POINT ( 'NONE',  ( 12.04999999999990834, 2.500000000000000000, 6.495190528383297135 ) ) ;
#102231=CARTESIAN_POINT ( 'NONE',  ( 0.5999999999999555689, 2.500000000000000000, 4.676537180435972552 ) ) ;
#102232=EDGE_CURVE ( 'NONE', #57293, #21757, #3343, .T. ) ;
#102233=ORIENTED_EDGE ( 'NONE', *, *, #129605, .T. ) ;
#102234=ORIENTED_EDGE ( 'NONE', *, *, #124509, .T. ) ;
#102237=VECTOR ( 'NONE', #112915, 1000.000000000000000 ) ;
#102238=DIRECTION ( 'NONE',  ( -0.000000000000000000, 1.000000000000000000, -0.000000000000000000 ) ) ;
#102241=DIRECTION ( 'NONE',  ( 0.000000000000000000, -0.000000000000000000, 1.000000000000000000 ) ) ;
#102242=CARTESIAN_POINT ( 'NONE',  ( -0.4500000000000397571, 2.500000000000000000, -2.265063509461101798 ) ) ;
#102243=DIRECTION ( 'NONE',  ( 0.000000000000000000, 0.000000000000000000, -1.000000000000000000 ) ) ;
#102244=DIRECTION ( 'NONE',  ( 0.000000000000000000, -0.9999939076577903929, 0.003490651415223739937 ) ) ;
#102245=DIRECTION ( 'NONE',  ( 0.000000000000000000, 1.000000000000000000, 0.000000000000000000 ) ) ;
#102246=AXIS2_PLACEMENT_3D ( 'NONE', #14675, #63150, #84721 ) ;
#102247=ORIENTED_EDGE ( 'NONE', *, *, #22729, .F. ) ;
#102250=CONICAL_SURFACE ( 'NONE', #112715, 0.09999999999999999167, 0.003490658503988666988 ) ;
#102251=VERTEX_POINT ( 'NONE', #121819 ) ;
#102252=PLANE ( 'NONE',  #62155 ) ;
#102253=CARTESIAN_POINT ( 'NONE',  ( -7.100000000000013856, 2.500000000000000000, 5.022947341949748790 ) ) ;
#102254=DIRECTION ( 'NONE',  ( 0.000000000000000000, 0.000000000000000000, 1.000000000000000000 ) ) ;
#102255=CIRCLE ( 'NONE', #64589, 0.1000000000000002554 ) ;
#102256=ORIENTED_EDGE ( 'NONE', *, *, #83534, .T. ) ;
#102257=VERTEX_POINT ( 'NONE', #53730 ) ;
#102258=FACE_BOUND ( 'NONE', #6897, .T. ) ;
#102259=ORIENTED_EDGE ( 'NONE', *, *, #31418, .F. ) ;
#102260=DIRECTION ( 'NONE',  ( 0.000000000000000000, 0.000000000000000000, 1.000000000000000000 ) ) ;
#102261=DIRECTION ( 'NONE',  ( 0.000000000000000000, 0.000000000000000000, -1.000000000000000000 ) ) ;
#102262=DIRECTION ( 'NONE',  ( 0.000000000000000000, -0.000000000000000000, 1.000000000000000000 ) ) ;
#102263=AXIS2_PLACEMENT_3D ( 'NONE', #24721, #43737, #33270 ) ;
#102264=CARTESIAN_POINT ( 'NONE',  ( 6.649999999999928413, 2.500000000000000000, 1.372243186433545370 ) ) ;
#102265=DIRECTION ( 'NONE',  ( -0.000000000000000000, 1.000000000000000000, -0.000000000000000000 ) ) ;
#102266=CARTESIAN_POINT ( 'NONE',  ( -3.750000000000029310, 2.500000000000000000, -7.188010851410854052 ) ) ;
#102267=CARTESIAN_POINT ( 'NONE',  ( 9.199999999999919353, 12.50000000000000000, 0.06509327318403515528 ) ) ;
#102268=DIRECTION ( 'NONE',  ( -4.274815082592931898E-19, -0.9999939076577903929, -0.003490651415223739937 ) ) ;
#102269=DIRECTION ( 'NONE',  ( -0.000000000000000000, -1.000000000000000000, -0.000000000000000000 ) ) ;
#102270=DIRECTION ( 'NONE',  ( 0.000000000000000000, 1.000000000000000000, 0.000000000000000000 ) ) ;
#102271=FACE_OUTER_BOUND ( 'NONE', #73909, .T. ) ;
#102272=ADVANCED_FACE ( 'NONE', ( #32823 ), #127746, .T. ) ;
#102273=ORIENTED_EDGE ( 'NONE', *, *, #101908, .T. ) ;
#102274=VERTEX_POINT ( 'NONE', #64830 ) ;
#102275=EDGE_LOOP ( 'NONE', ( #40547, #77314 ) ) ;
#102276=DIRECTION ( 'NONE',  ( -0.000000000000000000, 1.000000000000000000, -0.000000000000000000 ) ) ;
#102277=VERTEX_POINT ( 'NONE', #22359 ) ;
#102278=CARTESIAN_POINT ( 'NONE',  ( 12.89999999999990266, 2.500000000000000000, -5.022947341949754119 ) ) ;
#102279=AXIS2_PLACEMENT_3D ( 'NONE', #104958, #5474, #85341 ) ;
#102280=DIRECTION ( 'NONE',  ( -0.000000000000000000, 1.000000000000000000, -0.000000000000000000 ) ) ;
#102281=ORIENTED_EDGE ( 'NONE', *, *, #34648, .F. ) ;
#102282=VERTEX_POINT ( 'NONE', #3976 ) ;
#102283=ORIENTED_EDGE ( 'NONE', *, *, #77731, .T. ) ;
#102284=DIRECTION ( 'NONE',  ( 0.000000000000000000, 1.000000000000000000, 0.000000000000000000 ) ) ;
#102285=AXIS2_PLACEMENT_3D ( 'NONE', #60807, #62750, #123575 ) ;
#102286=AXIS2_PLACEMENT_3D ( 'NONE', #48387, #8439, #79154 ) ;
#102287=CARTESIAN_POINT ( 'NONE',  ( 4.399999999999937295, 12.50000000000000000, 4.676537180435972552 ) ) ;
#102288=FACE_OUTER_BOUND ( 'NONE', #116984, .T. ) ;
#102290=EDGE_CURVE ( 'NONE', #102251, #86684, #44117, .T. ) ;
#102291=CARTESIAN_POINT ( 'NONE',  ( -1.900000000000034106, 2.500000000000000000, -4.083716857408426826 ) ) ;
#102292=EDGE_CURVE ( 'NONE', #111573, #54835, #4589, .T. ) ;
#102293=EDGE_LOOP ( 'NONE', ( #3989, #110492 ) ) ;
#102294=CIRCLE ( 'NONE', #77238, 0.1000000000000002554 ) ;
#102295=VECTOR ( 'NONE', #77025, 1000.000000000000000 ) ;
#102296=CARTESIAN_POINT ( 'NONE',  ( -3.950000000000029932, 12.50000000000000000, -6.148780366869526226 ) ) ;
#102297=ORIENTED_EDGE ( 'NONE', *, *, #35571, .T. ) ;
#102298=VECTOR ( 'NONE', #35479, 1000.000000000000000 ) ;
#102299=EDGE_LOOP ( 'NONE', ( #89188, #23615 ) ) ;
#102300=EDGE_LOOP ( 'NONE', ( #31348, #53863 ) ) ;
#102301=DIRECTION ( 'NONE',  ( -0.000000000000000000, -1.000000000000000000, -0.000000000000000000 ) ) ;
#102302=ORIENTED_EDGE ( 'NONE', *, *, #14671, .T. ) ;
#102303=EDGE_CURVE ( 'NONE', #124247, #75500, #98478, .T. ) ;
#102304=ORIENTED_EDGE ( 'NONE', *, *, #78094, .F. ) ;
#102305=VERTEX_POINT ( 'NONE', #103479 ) ;
#102306=AXIS2_PLACEMENT_3D ( 'NONE', #80160, #99806, #50696 ) ;
#102308=CIRCLE ( 'NONE', #114891, 0.1000000000000002554 ) ;
#102309=PLANE ( 'NONE',  #101988 ) ;
#102310=CARTESIAN_POINT ( 'NONE',  ( 6.649999999999929301, 2.500000000000000000, 6.495190528383297135 ) ) ;
#102311=CIRCLE ( 'NONE', #54272, 0.1000000000000002554 ) ;
#102312=CARTESIAN_POINT ( 'NONE',  ( -9.600000000000008527, 12.50000000000000000, -5.022947341949749678 ) ) ;
#102313=DIRECTION ( 'NONE',  ( 0.000000000000000000, 1.000000000000000000, 0.000000000000000000 ) ) ;
#102314=CARTESIAN_POINT ( 'NONE',  ( 9.349999999999919709, 2.500000000000000000, 1.818653347947321475 ) ) ;
#102315=CARTESIAN_POINT ( 'NONE',  ( 5.849999999999933031, 12.50000000000000000, -1.472243186433550122 ) ) ;
#102316=ORIENTED_EDGE ( 'NONE', *, *, #5818, .F. ) ;
#102317=FACE_OUTER_BOUND ( 'NONE', #52470, .T. ) ;
#102318=ORIENTED_EDGE ( 'NONE', *, *, #129283, .T. ) ;
#102319=DIRECTION ( 'NONE',  ( -4.274815082592931898E-19, -0.9999939076577903929, -0.003490651415223739937 ) ) ;
#102320=CIRCLE ( 'NONE', #112784, 0.06509327318403743123 ) ;
#102321=VERTEX_POINT ( 'NONE', #34756 ) ;
#102322=CARTESIAN_POINT ( 'NONE',  ( 0.1999999999999576006, 12.50000000000000000, -4.741630453620016006 ) ) ;
#102323=VERTEX_POINT ( 'NONE', #83204 ) ;
#102325=EDGE_CURVE ( 'NONE', #74675, #33200, #112656, .T. ) ;
#102326=DIRECTION ( 'NONE',  ( -0.000000000000000000, -1.000000000000000000, -0.000000000000000000 ) ) ;
#102327=VERTEX_POINT ( 'NONE', #64188 ) ;
#102328=EDGE_LOOP ( 'NONE', ( #2366, #52599, #92780, #2452 ) ) ;
#102329=CARTESIAN_POINT ( 'NONE',  ( -2.499999999999996447, 2.500000000000000000, 4.330127018922196314 ) ) ;
#102330=DIRECTION ( 'NONE',  ( 0.000000000000000000, -0.000000000000000000, 1.000000000000000000 ) ) ;
#102331=EDGE_CURVE ( 'NONE', #81523, #51798, #67162, .T. ) ;
#102332=DIRECTION ( 'NONE',  ( 0.000000000000000000, 0.000000000000000000, -1.000000000000000000 ) ) ;
#102333=FACE_OUTER_BOUND ( 'NONE', #49626, .T. ) ;
#102334=AXIS2_PLACEMENT_3D ( 'NONE', #103599, #51923, #91840 ) ;
#102335=ADVANCED_FACE ( 'NONE', ( #91723 ), #93660, .T. ) ;
#102336=CARTESIAN_POINT ( 'NONE',  ( 9.599999999999914380, 2.500000000000000000, 4.330127018922196314 ) ) ;
#102337=ORIENTED_EDGE ( 'NONE', *, *, #92082, .T. ) ;
#102338=DIRECTION ( 'NONE',  ( -0.000000000000000000, 1.000000000000000000, -0.000000000000000000 ) ) ;
#102339=EDGE_CURVE ( 'NONE', #89915, #34182, #27371, .T. ) ;
#102340=ADVANCED_FACE ( 'NONE', ( #33464 ), #50470, .T. ) ;
#102341=CONICAL_SURFACE ( 'NONE', #35442, 0.1000000000000002554, 0.003490658503988666988 ) ;
#102342=EDGE_CURVE ( 'NONE', #62801, #123416, #46260, .T. ) ;
#102343=ORIENTED_EDGE ( 'NONE', *, *, #26649, .T. ) ;
#102344=PLANE ( 'NONE',  #13015 ) ;
#102345=CARTESIAN_POINT ( 'NONE',  ( -7.950000000000016165, 2.500000000000000000, -6.495190528383297135 ) ) ;
#102346=AXIS2_PLACEMENT_3D ( 'NONE', #68515, #99283, #46965 ) ;
#102347=CIRCLE ( 'NONE', #62639, 0.06509327318403741736 ) ;
#102348=ADVANCED_FACE ( 'NONE', ( #115869 ), #123615, .T. ) ;
#102349=CIRCLE ( 'NONE', #20866, 0.06509327318403745899 ) ;
#102350=CARTESIAN_POINT ( 'NONE',  ( 6.449999999999931788, 2.500000000000000000, 6.148780366869520009 ) ) ;
#102351=LINE ( 'NONE', #91879, #122139 ) ;
#102352=PLANE ( 'NONE',  #113467 ) ;
#102353=DIRECTION ( 'NONE',  ( 0.000000000000000000, 0.000000000000000000, 1.000000000000000000 ) ) ;
#102354=CARTESIAN_POINT ( 'NONE',  ( 13.74999999999993072, 2.500000000000000000, -2.165063509461101710 ) ) ;
#102355=ORIENTED_EDGE ( 'NONE', *, *, #39428, .T. ) ;
#102356=EDGE_CURVE ( 'NONE', #107669, #87317, #100549, .T. ) ;
#102357=AXIS2_PLACEMENT_3D ( 'NONE', #6330, #118896, #16796 ) ;
#102358=AXIS2_PLACEMENT_3D ( 'NONE', #15403, #55352, #25890 ) ;
#102359=DIRECTION ( 'NONE',  ( 0.000000000000000000, 0.000000000000000000, -1.000000000000000000 ) ) ;
#102360=LINE ( 'NONE', #72893, #67253 ) ;
#102361=CARTESIAN_POINT ( 'NONE',  ( -8.150000000000012790, 2.500000000000000000, 1.818653347947321475 ) ) ;
#102362=ORIENTED_EDGE ( 'NONE', *, *, #121513, .T. ) ;
#102363=ORIENTED_EDGE ( 'NONE', *, *, #37209, .F. ) ;
#102364=CARTESIAN_POINT ( 'NONE',  ( -12.09999999999999432, 2.500000000000000000, 5.022947341949748790 ) ) ;
#102365=ORIENTED_EDGE ( 'NONE', *, *, #100227, .F. ) ;
#102366=EDGE_LOOP ( 'NONE', ( #49001, #75027 ) ) ;
#102367=FACE_OUTER_BOUND ( 'NONE', #41834, .T. ) ;
#102368=AXIS2_PLACEMENT_3D ( 'NONE', #2101, #825, #11285 ) ;
#102369=ORIENTED_EDGE ( 'NONE', *, *, #65125, .F. ) ;
#102370=CARTESIAN_POINT ( 'NONE',  ( 19.21290572970430333, -2.587129408759125226, -2.394140119533374911 ) ) ;
#102371=DIRECTION ( 'NONE',  ( 0.000000000000000000, 0.000000000000000000, -1.000000000000000000 ) ) ;
#102372=FACE_OUTER_BOUND ( 'NONE', #2060, .T. ) ;
#102373=ORIENTED_EDGE ( 'NONE', *, *, #25813, .F. ) ;
#102374=CIRCLE ( 'NONE', #62669, 0.09999999999999999167 ) ;
#102375=CARTESIAN_POINT ( 'NONE',  ( -3.350000000000029399, 12.50000000000000000, 6.495190528383297135 ) ) ;
#102376=CONICAL_SURFACE ( 'NONE', #45947, 0.1000000000000000472, 0.003490658503988666988 ) ;
#102377=DIRECTION ( 'NONE',  ( 0.000000000000000000, 0.000000000000000000, -1.000000000000000000 ) ) ;
#102378=AXIS2_PLACEMENT_3D ( 'NONE', #108120, #8611, #9925 ) ;
#102379=ORIENTED_EDGE ( 'NONE', *, *, #62035, .F. ) ;
#102380=AXIS2_PLACEMENT_3D ( 'NONE', #21996, #69129, #71715 ) ;
#102381=AXIS2_PLACEMENT_3D ( 'NONE', #6616, #26947, #76689 ) ;
#102382=ADVANCED_FACE ( 'NONE', ( #127624 ), #23272, .T. ) ;
#102383=ORIENTED_EDGE ( 'NONE', *, *, #80457, .T. ) ;
#102384=ORIENTED_EDGE ( 'NONE', *, *, #67373, .F. ) ;
#102385=CARTESIAN_POINT ( 'NONE',  ( 7.899999999999924860, 12.50000000000000000, 5.022947341949748790 ) ) ;
#102386=DIRECTION ( 'NONE',  ( 0.000000000000000000, 1.000000000000000000, 0.000000000000000000 ) ) ;
#102387=FACE_BOUND ( 'NONE', #5716, .T. ) ;
#102388=ORIENTED_EDGE ( 'NONE', *, *, #48959, .T. ) ;
#102389=AXIS2_PLACEMENT_3D ( 'NONE', #112049, #11904, #11253 ) ;
#102390=DIRECTION ( 'NONE',  ( 0.000000000000000000, -0.000000000000000000, 1.000000000000000000 ) ) ;
#102391=DIRECTION ( 'NONE',  ( 0.000000000000000000, 1.000000000000000000, 0.000000000000000000 ) ) ;
#102392=ORIENTED_EDGE ( 'NONE', *, *, #92132, .T. ) ;
#102393=EDGE_CURVE ( 'NONE', #51917, #59583, #26206, .T. ) ;
#102394=DIRECTION ( 'NONE',  ( 0.000000000000000000, 0.000000000000000000, 1.000000000000000000 ) ) ;
#102395=DIRECTION ( 'NONE',  ( 0.000000000000000000, 1.000000000000000000, 0.000000000000000000 ) ) ;
#102396=AXIS2_PLACEMENT_3D ( 'NONE', #70807, #110092, #32839 ) ;
#102397=DIRECTION ( 'NONE',  ( -4.274815082592931898E-19, -0.9999939076577903929, -0.003490651415223739937 ) ) ;
#102398=CARTESIAN_POINT ( 'NONE',  ( -9.600000000000006750, 12.50000000000000000, 5.022947341949748790 ) ) ;
#102399=DIRECTION ( 'NONE',  ( 0.000000000000000000, 0.000000000000000000, 1.000000000000000000 ) ) ;
#102400=CARTESIAN_POINT ( 'NONE',  ( -9.200000000000006395, 12.50000000000000000, 4.330127018922196314 ) ) ;
#102401=DIRECTION ( 'NONE',  ( -0.000000000000000000, -1.000000000000000000, -0.000000000000000000 ) ) ;
#102402=AXIS2_PLACEMENT_3D ( 'NONE', #37152, #27300, #85589 ) ;
#102403=ORIENTED_EDGE ( 'NONE', *, *, #106338, .T. ) ;
#102404=VERTEX_POINT ( 'NONE', #57607 ) ;
#102405=VERTEX_POINT ( 'NONE', #85755 ) ;
#102406=ORIENTED_EDGE ( 'NONE', *, *, #49462, .T. ) ;
#102407=CONICAL_SURFACE ( 'NONE', #106508, 0.1000000000000000472, 0.003490658503988666988 ) ;
#102408=DIRECTION ( 'NONE',  ( -0.000000000000000000, 1.000000000000000000, -0.000000000000000000 ) ) ;
#102409=LINE ( 'NONE', #82117, #118890 ) ;
#102410=DIRECTION ( 'NONE',  ( 0.000000000000000000, -0.9999939076577903929, 0.003490651415223739937 ) ) ;
#102411=EDGE_LOOP ( 'NONE', ( #21949, #54618, #76421, #108183 ) ) ;
#102412=FACE_BOUND ( 'NONE', #113960, .T. ) ;
#102413=PLANE ( 'NONE',  #100217 ) ;
#102414=CARTESIAN_POINT ( 'NONE',  ( -1.450000000000035927, 2.500000000000000000, -1.818653347947326138 ) ) ;
#102416=FACE_OUTER_BOUND ( 'NONE', #31162, .T. ) ;
#102417=DIRECTION ( 'NONE',  ( 0.000000000000000000, 1.000000000000000000, 0.000000000000000000 ) ) ;
#102419=CARTESIAN_POINT ( 'NONE',  ( 10.84999999999991260, 2.500000000000000000, -2.757883832488654097 ) ) ;
#102420=DIRECTION ( 'NONE',  ( 0.000000000000000000, 0.000000000000000000, -1.000000000000000000 ) ) ;
#102421=DIRECTION ( 'NONE',  ( 0.000000000000000000, 1.000000000000000000, 0.000000000000000000 ) ) ;
#102422=EDGE_LOOP ( 'NONE', ( #83669, #87365 ) ) ;
#102423=EDGE_CURVE ( 'NONE', #110342, #27555, #75496, .T. ) ;
#102424=EDGE_LOOP ( 'NONE', ( #78704, #31080 ) ) ;
#102425=EDGE_LOOP ( 'NONE', ( #3704, #45741 ) ) ;
#102426=VERTEX_POINT ( 'NONE', #26848 ) ;
#102427=ORIENTED_EDGE ( 'NONE', *, *, #112739, .F. ) ;
#102428=VERTEX_POINT ( 'NONE', #45849 ) ;
#102429=DIRECTION ( 'NONE',  ( -0.000000000000000000, -1.000000000000000000, -0.000000000000000000 ) ) ;
#102430=AXIS2_PLACEMENT_3D ( 'NONE', #18237, #68627, #129521 ) ;
#102431=ORIENTED_EDGE ( 'NONE', *, *, #42125, .F. ) ;
#102432=VERTEX_POINT ( 'NONE', #5259 ) ;
#102433=EDGE_CURVE ( 'NONE', #114003, #57219, #96420, .T. ) ;
#102434=AXIS2_PLACEMENT_3D ( 'NONE', #17302, #56597, #96517 ) ;
#102435=CARTESIAN_POINT ( 'NONE',  ( 4.149999999999941735, 2.500000000000000000, -7.188010851410854052 ) ) ;
#102436=AXIS2_PLACEMENT_3D ( 'NONE', #97867, #48136, #88021 ) ;
#102437=CARTESIAN_POINT ( 'NONE',  ( 13.80679872386857276, -1.499999999999904077, 7.946844943073641865 ) ) ;
#102438=CARTESIAN_POINT ( 'NONE',  ( -2.300000000000033129, 2.500000000000000000, 4.083716857408420609 ) ) ;
#102439=DIRECTION ( 'NONE',  ( 0.000000000000000000, -0.000000000000000000, 1.000000000000000000 ) ) ;
#102440=ADVANCED_FACE ( 'NONE', ( #36025 ), #58793, .T. ) ;
#102441=EDGE_CURVE ( 'NONE', #14735, #42734, #4379, .T. ) ;
#102442=ORIENTED_EDGE ( 'NONE', *, *, #27397, .F. ) ;
#102443=DIRECTION ( 'NONE',  ( 0.000000000000000000, 1.000000000000000000, 0.000000000000000000 ) ) ;
#102444=CIRCLE ( 'NONE', #100388, 0.1000000000000000472 ) ;
#102445=AXIS2_PLACEMENT_3D ( 'NONE', #15738, #54379, #114583 ) ;
#102446=ORIENTED_EDGE ( 'NONE', *, *, #1160, .F. ) ;
#102447=ORIENTED_EDGE ( 'NONE', *, *, #48257, .F. ) ;
#102448=DIRECTION ( 'NONE',  ( -4.274815082592931898E-19, -0.9999939076577903929, -0.003490651415223739937 ) ) ;
#102449=EDGE_CURVE ( 'NONE', #101033, #64350, #77556, .T. ) ;
#102450=DIRECTION ( 'NONE',  ( 0.000000000000000000, 0.000000000000000000, 1.000000000000000000 ) ) ;
#102451=EDGE_CURVE ( 'NONE', #20100, #106061, #48323, .T. ) ;
#102452=ORIENTED_EDGE ( 'NONE', *, *, #51656, .F. ) ;
#102453=ORIENTED_EDGE ( 'NONE', *, *, #25311, .T. ) ;
#102454=DIRECTION ( 'NONE',  ( -0.000000000000000000, 1.000000000000000000, -0.000000000000000000 ) ) ;
#102455=DIRECTION ( 'NONE',  ( 0.000000000000000000, 0.000000000000000000, 1.000000000000000000 ) ) ;
#102456=FACE_OUTER_BOUND ( 'NONE', #55344, .T. ) ;
#102457=DIRECTION ( 'NONE',  ( -0.000000000000000000, -1.000000000000000000, -0.000000000000000000 ) ) ;
#102458=CARTESIAN_POINT ( 'NONE',  ( -6.650000000000014566, 2.500000000000000000, 6.495190528383297135 ) ) ;
#102459=ORIENTED_EDGE ( 'NONE', *, *, #128163, .T. ) ;
#102460=CARTESIAN_POINT ( 'NONE',  ( 10.19999999999991580, 12.50000000000000000, -0.3464101615137783474 ) ) ;
#102461=AXIS2_PLACEMENT_3D ( 'NONE', #26149, #97460, #45794 ) ;
#102462=VECTOR ( 'NONE', #80411, 1000.000000000000000 ) ;
#102463=ORIENTED_EDGE ( 'NONE', *, *, #82727, .F. ) ;
#102464=CARTESIAN_POINT ( 'NONE',  ( 87.50000000000001421, 3.974992050023848922, -6.359987280038160051 ) ) ;
#102465=LINE ( 'NONE', #54013, #12853 ) ;
#102466=CARTESIAN_POINT ( 'NONE',  ( -7.700000000000016165, 2.500000000000000000, -3.883716857408426648 ) ) ;
#102467=DIRECTION ( 'NONE',  ( -0.000000000000000000, 1.000000000000000000, -0.000000000000000000 ) ) ;
#102468=CARTESIAN_POINT ( 'NONE',  ( -7.499999999999980460, 2.500000000000000000, -4.330127018922201643 ) ) ;
#102469=ORIENTED_EDGE ( 'NONE', *, *, #111776, .T. ) ;
#102470=CIRCLE ( 'NONE', #79496, 0.06509327318403745899 ) ;
#102471=CARTESIAN_POINT ( 'NONE',  ( 11.44999999999991047, 12.50000000000000000, -2.511473670974877948 ) ) ;
#102472=PLANE ( 'NONE',  #79982 ) ;
#102473=ORIENTED_EDGE ( 'NONE', *, *, #126674, .T. ) ;
#102474=EDGE_LOOP ( 'NONE', ( #86109, #106914 ) ) ;
#102475=ORIENTED_EDGE ( 'NONE', *, *, #74269, .T. ) ;
#102476=DIRECTION ( 'NONE',  ( -0.000000000000000000, -1.000000000000000000, -0.000000000000000000 ) ) ;
#102477=DIRECTION ( 'NONE',  ( 0.000000000000000000, 1.000000000000000000, 0.000000000000000000 ) ) ;
#102479=AXIS2_PLACEMENT_3D ( 'NONE', #9664, #129470, #79688 ) ;
#102480=CARTESIAN_POINT ( 'NONE',  ( -5.000000000000022204, 2.500000000000000000, 3.637306695894644726 ) ) ;
#102481=DIRECTION ( 'NONE',  ( 0.000000000000000000, -0.9999939076577903929, 0.003490651415223739937 ) ) ;
#102482=EDGE_CURVE ( 'NONE', #46048, #21956, #21132, .T. ) ;
#102483=CIRCLE ( 'NONE', #18931, 0.09999999999999982514 ) ;
#102484=CARTESIAN_POINT ( 'NONE',  ( 10.84999999999991260, 12.50000000000000000, -2.857883832488653741 ) ) ;
#102485=PLANE ( 'NONE',  #562 ) ;
#102487=ADVANCED_FACE ( 'NONE', ( #95591 ), #2330, .T. ) ;
#102488=EDGE_CURVE ( 'NONE', #114610, #109551, #65021, .T. ) ;
#102489=VECTOR ( 'NONE', #24136, 1000.000000000000000 ) ;
#102490=ADVANCED_FACE ( 'NONE', ( #126987 ), #17662, .T. ) ;
#102491=CARTESIAN_POINT ( 'NONE',  ( -11.64999999999999680, 2.500000000000000000, 2.957883832488649389 ) ) ;
#102492=ORIENTED_EDGE ( 'NONE', *, *, #58004, .T. ) ;
#102493=EDGE_CURVE ( 'NONE', #102028, #56755, #92225, .T. ) ;
#102494=AXIS2_PLACEMENT_3D ( 'NONE', #128978, #127026, #68082 ) ;
#102495=DIRECTION ( 'NONE',  ( 0.000000000000000000, 1.000000000000000000, 0.000000000000000000 ) ) ;
#102496=DIRECTION ( 'NONE',  ( 0.000000000000000000, 1.000000000000000000, 0.000000000000000000 ) ) ;
#102497=CARTESIAN_POINT ( 'NONE',  ( -0.6000000000000323963, 12.50000000000000000, 0.3464101615137759604 ) ) ;
#102498=PLANE ( 'NONE',  #104395 ) ;
#102499=ORIENTED_EDGE ( 'NONE', *, *, #91357, .F. ) ;
#102500=ADVANCED_FACE ( 'NONE', ( #7839 ), #97514, .T. ) ;
#102501=DIRECTION ( 'NONE',  ( 0.000000000000000000, -0.000000000000000000, 1.000000000000000000 ) ) ;
#102502=EDGE_CURVE ( 'NONE', #66522, #63978, #118442, .T. ) ;
#102503=DIRECTION ( 'NONE',  ( 0.000000000000000000, -0.9999939076577903929, 0.003490651415223739937 ) ) ;
#102504=CARTESIAN_POINT ( 'NONE',  ( 6.899999999999928413, 2.500000000000000000, 3.983716857408420964 ) ) ;
#102505=ORIENTED_EDGE ( 'NONE', *, *, #50400, .T. ) ;
#102506=VERTEX_POINT ( 'NONE', #19609 ) ;
#102507=DIRECTION ( 'NONE',  ( 0.000000000000000000, 1.000000000000000000, 0.000000000000000000 ) ) ;
#102508=ORIENTED_EDGE ( 'NONE', *, *, #55509, .F. ) ;
#102509=ORIENTED_EDGE ( 'NONE', *, *, #36877, .F. ) ;
#102510=CARTESIAN_POINT ( 'NONE',  ( -4.150000000000028777, 2.500000000000000000, -5.802370205355749988 ) ) ;
#102511=AXIS2_PLACEMENT_3D ( 'NONE', #112438, #20830, #22138 ) ;
#102512=CARTESIAN_POINT ( 'NONE',  ( -2.950000000000033484, 12.50000000000000000, -6.560283801567339701 ) ) ;
#102513=CARTESIAN_POINT ( 'NONE',  ( -12.69999999999999396, 2.500000000000000000, -3.883716857408423984 ) ) ;
#102514=DIRECTION ( 'NONE',  ( 0.000000000000000000, 1.000000000000000000, 0.000000000000000000 ) ) ;
#102515=EDGE_LOOP ( 'NONE', ( #59448, #115400 ) ) ;
#102516=CIRCLE ( 'NONE', #2165, 0.06509327318403745899 ) ;
#102517=CARTESIAN_POINT ( 'NONE',  ( -9.550000000000002487, 12.50000000000000000, 6.560283801567334372 ) ) ;
#102519=ORIENTED_EDGE ( 'NONE', *, *, #41005, .T. ) ;
#102520=CARTESIAN_POINT ( 'NONE',  ( 17.48307833624052066, 2.102402844588128428, 4.293715869771017601 ) ) ;
#102521=DIRECTION ( 'NONE',  ( 0.000000000000000000, -0.000000000000000000, 1.000000000000000000 ) ) ;
#102522=VERTEX_POINT ( 'NONE', #90928 ) ;
#102523=EDGE_LOOP ( 'NONE', ( #98886, #26844 ) ) ;
#102524=ORIENTED_EDGE ( 'NONE', *, *, #116953, .F. ) ;
#102525=VERTEX_POINT ( 'NONE', #70006 ) ;
#102526=PLANE ( 'NONE',  #64987 ) ;
#102527=CARTESIAN_POINT ( 'NONE',  ( -10.85000000000000142, 2.500000000000000000, -6.395190528383298378 ) ) ;
#102528=CARTESIAN_POINT ( 'NONE',  ( -3.350000000000028511, 2.500000000000000000, 2.957883832488649389 ) ) ;
#102529=FACE_BOUND ( 'NONE', #104855, .T. ) ;
#102532=DIRECTION ( 'NONE',  ( -0.000000000000000000, 1.000000000000000000, -0.000000000000000000 ) ) ;
#102533=DIRECTION ( 'NONE',  ( 0.000000000000000000, -0.000000000000000000, 1.000000000000000000 ) ) ;
#102534=EDGE_CURVE ( 'NONE', #19850, #122843, #125668, .T. ) ;
#102535=DIRECTION ( 'NONE',  ( 0.000000000000000000, 1.000000000000000000, 0.000000000000000000 ) ) ;
#102536=DIRECTION ( 'NONE',  ( -0.7336674352944539956, 0.000000000000000000, -0.6795087154617358571 ) ) ;
#102537=LINE ( 'NONE', #120889, #103578 ) ;
#102538=VECTOR ( 'NONE', #78332, 1000.000000000000000 ) ;
#102539=CARTESIAN_POINT ( 'NONE',  ( -1.650000000000035216, 2.500000000000000000, -1.472243186433550122 ) ) ;
#102540=VERTEX_POINT ( 'NONE', #59568 ) ;
#102541=EDGE_LOOP ( 'NONE', ( #55088, #113017, #18750, #75542 ) ) ;
#102542=VERTEX_POINT ( 'NONE', #128288 ) ;
#102543=VERTEX_POINT ( 'NONE', #49090 ) ;
#102544=ORIENTED_EDGE ( 'NONE', *, *, #85776, .F. ) ;
#102546=DIRECTION ( 'NONE',  ( 0.000000000000000000, 0.000000000000000000, 1.000000000000000000 ) ) ;
#102547=ORIENTED_EDGE ( 'NONE', *, *, #32460, .T. ) ;
#102548=FACE_BOUND ( 'NONE', #2491, .T. ) ;
#102549=CIRCLE ( 'NONE', #48271, 0.06509327318403745899 ) ;
#102550=FACE_OUTER_BOUND ( 'NONE', #14713, .T. ) ;
#102551=EDGE_LOOP ( 'NONE', ( #44040, #25787, #42222, #63946 ) ) ;
#102552=CARTESIAN_POINT ( 'NONE',  ( 6.449999999999931788, 2.500000000000000000, 6.048780366869520364 ) ) ;
#102553=FACE_OUTER_BOUND ( 'NONE', #124998, .T. ) ;
#102554=DIRECTION ( 'NONE',  ( 0.000000000000000000, -0.9999939076577903929, 0.003490651415223739937 ) ) ;
#102555=ORIENTED_EDGE ( 'NONE', *, *, #65579, .F. ) ;
#102556=CARTESIAN_POINT ( 'NONE',  ( 1.899999999999949507, 2.500000000000000000, 4.676537180435972552 ) ) ;
#102557=CIRCLE ( 'NONE', #56581, 0.1000000000000002554 ) ;
#102558=ORIENTED_EDGE ( 'NONE', *, *, #87417, .F. ) ;
#102559=CIRCLE ( 'NONE', #6391, 0.06509327318403745899 ) ;
#102560=ORIENTED_EDGE ( 'NONE', *, *, #25263, .F. ) ;
#102561=EDGE_LOOP ( 'NONE', ( #119821, #126170, #71454, #109851 ) ) ;
#102562=PLANE ( 'NONE',  #77895 ) ;
#102563=CARTESIAN_POINT ( 'NONE',  ( -5.600000000000020073, 2.500000000000000000, 3.983716857408420964 ) ) ;
#102564=CARTESIAN_POINT ( 'NONE',  ( -11.69999999999999929, 2.500000000000000000, 0.1000000000000017403 ) ) ;
#102565=VERTEX_POINT ( 'NONE', #98797 ) ;
#102566=CARTESIAN_POINT ( 'NONE',  ( 2.899999999999943956, 12.50000000000000000, 4.330127018922196314 ) ) ;
#102567=EDGE_CURVE ( 'NONE', #81614, #20666, #11056, .T. ) ;
#102568=DIRECTION ( 'NONE',  ( 0.000000000000000000, 0.000000000000000000, 1.000000000000000000 ) ) ;
#102569=CARTESIAN_POINT ( 'NONE',  ( 4.149999999999939959, 2.500000000000000000, -2.265063509461101798 ) ) ;
#102570=CONICAL_SURFACE ( 'NONE', #87890, 0.09999999999999982514, 0.003490658503988666988 ) ;
#102572=ORIENTED_EDGE ( 'NONE', *, *, #74352, .T. ) ;
#102573=EDGE_CURVE ( 'NONE', #65666, #39808, #18307, .T. ) ;
#102574=DIRECTION ( 'NONE',  ( -0.000000000000000000, -1.000000000000000000, -0.000000000000000000 ) ) ;
#102575=ADVANCED_FACE ( 'NONE', ( #89641 ), #73534, .T. ) ;
#102576=ORIENTED_EDGE ( 'NONE', *, *, #53407, .F. ) ;
#102577=FACE_OUTER_BOUND ( 'NONE', #104823, .T. ) ;
#102578=ORIENTED_EDGE ( 'NONE', *, *, #77326, .F. ) ;
#102579=ORIENTED_EDGE ( 'NONE', *, *, #123015, .T. ) ;
#102580=DIRECTION ( 'NONE',  ( 0.000000000000000000, 0.000000000000000000, 1.000000000000000000 ) ) ;
#102581=CARTESIAN_POINT ( 'NONE',  ( 6.049999999999932321, 12.50000000000000000, -1.818653347947326138 ) ) ;
#102582=EDGE_CURVE ( 'NONE', #103695, #50900, #48414, .T. ) ;
#102583=EDGE_CURVE ( 'NONE', #10632, #23431, #25408, .T. ) ;
#102584=LINE ( 'NONE', #121578, #113490 ) ;
#102585=EDGE_CURVE ( 'NONE', #1863, #101462, #17077, .T. ) ;
#102586=DIRECTION ( 'NONE',  ( -4.274815082592931898E-19, -0.9999939076577903929, -0.003490651415223739937 ) ) ;
#102587=EDGE_CURVE ( 'NONE', #101787, #57283, #54657, .T. ) ;
#102588=DIRECTION ( 'NONE',  ( 0.000000000000000000, 1.000000000000000000, 0.000000000000000000 ) ) ;
#102589=EDGE_LOOP ( 'NONE', ( #62425, #30626 ) ) ;
#102590=ORIENTED_EDGE ( 'NONE', *, *, #99079, .T. ) ;
#102591=DIRECTION ( 'NONE',  ( 0.000000000000000000, 1.000000000000000000, 0.000000000000000000 ) ) ;
#102592=CARTESIAN_POINT ( 'NONE',  ( -10.40000000000000213, 2.500000000000000000, 4.330127018922196314 ) ) ;
#102593=CIRCLE ( 'NONE', #96328, 0.06509327318403745899 ) ;
#102594=DIRECTION ( 'NONE',  ( -0.000000000000000000, 1.000000000000000000, -0.000000000000000000 ) ) ;
#102595=EDGE_LOOP ( 'NONE', ( #107329, #111784 ) ) ;
#102596=ORIENTED_EDGE ( 'NONE', *, *, #72429, .T. ) ;
#102597=CONICAL_SURFACE ( 'NONE', #119323, 0.1000000000000000472, 0.003490658503988666988 ) ;
#102598=EDGE_CURVE ( 'NONE', #63617, #86820, #33835, .T. ) ;
#102599=DIRECTION ( 'NONE',  ( 0.000000000000000000, 1.000000000000000000, 0.000000000000000000 ) ) ;
#102600=ORIENTED_EDGE ( 'NONE', *, *, #126679, .T. ) ;
#102601=DIRECTION ( 'NONE',  ( 0.000000000000000000, 0.000000000000000000, 1.000000000000000000 ) ) ;
#102602=DIRECTION ( 'NONE',  ( 0.000000000000000000, -0.000000000000000000, 1.000000000000000000 ) ) ;
#102603=VECTOR ( 'NONE', #28297, 1000.000000000000000 ) ;
#102604=DIRECTION ( 'NONE',  ( -0.000000000000000000, -1.000000000000000000, -0.000000000000000000 ) ) ;
#102605=VERTEX_POINT ( 'NONE', #80484 ) ;
#102606=LINE ( 'NONE', #84253, #121326 ) ;
#102607=DIRECTION ( 'NONE',  ( -0.000000000000000000, 1.000000000000000000, -0.000000000000000000 ) ) ;
#102608=DIRECTION ( 'NONE',  ( 0.000000000000000000, 0.000000000000000000, 1.000000000000000000 ) ) ;
#102609=DIRECTION ( 'NONE',  ( 0.000000000000000000, 1.000000000000000000, 0.000000000000000000 ) ) ;
#102610=AXIS2_PLACEMENT_3D ( 'NONE', #67822, #29842, #27904 ) ;
#102611=CARTESIAN_POINT ( 'NONE',  ( 4.149999999999938183, 2.500000000000000000, 5.702370205355745014 ) ) ;
#102612=ORIENTED_EDGE ( 'NONE', *, *, #35367, .T. ) ;
#102613=CARTESIAN_POINT ( 'NONE',  ( 5.199999999999933564, 2.500000000000000000, 3.883716857408420431 ) ) ;
#102614=CARTESIAN_POINT ( 'NONE',  ( 48.67919755208251331, -3.179368040553702812, 5.083101272021607997 ) ) ;
#102615=ORIENTED_EDGE ( 'NONE', *, *, #42855, .F. ) ;
#102616=ORIENTED_EDGE ( 'NONE', *, *, #79472, .T. ) ;
#102617=ADVANCED_FACE ( 'NONE', ( #128943 ), #129589, .T. ) ;
#102619=DIRECTION ( 'NONE',  ( -0.000000000000000000, 1.000000000000000000, -0.000000000000000000 ) ) ;
#102620=CARTESIAN_POINT ( 'NONE',  ( 12.89999999999989733, 2.500000000000000000, -2.385244779468109755E-15 ) ) ;
#102621=DIRECTION ( 'NONE',  ( 0.000000000000000000, 0.000000000000000000, 1.000000000000000000 ) ) ;
#102622=CARTESIAN_POINT ( 'NONE',  ( -10.65000000000000213, 2.500000000000000000, 6.148780366869520009 ) ) ;
#102623=AXIS2_PLACEMENT_3D ( 'NONE', #115785, #26128, #66039 ) ;
#102624=CARTESIAN_POINT ( 'NONE',  ( 11.84999999999990727, 2.500000000000000000, 6.741600689897071952 ) ) ;
#102625=DIRECTION ( 'NONE',  ( 0.000000000000000000, 0.000000000000000000, -1.000000000000000000 ) ) ;
#102626=DIRECTION ( 'NONE',  ( 0.000000000000000000, -0.9999939076577903929, 0.003490651415223739937 ) ) ;
#102628=ADVANCED_FACE ( 'NONE', ( #71276 ), #119729, .T. ) ;
#102629=CARTESIAN_POINT ( 'NONE',  ( -8.150000000000014566, 12.50000000000000000, -6.083687093685483660 ) ) ;
#102630=AXIS2_PLACEMENT_3D ( 'NONE', #68028, #117753, #39249 ) ;
#102631=ORIENTED_EDGE ( 'NONE', *, *, #4619, .T. ) ;
#102633=ORIENTED_EDGE ( 'NONE', *, *, #50269, .F. ) ;
#102634=EDGE_CURVE ( 'NONE', #115112, #82663, #113254, .T. ) ;
#102635=ORIENTED_EDGE ( 'NONE', *, *, #91982, .F. ) ;
#102636=EDGE_LOOP ( 'NONE', ( #77976, #56934, #91, #77698 ) ) ;
#102637=ADVANCED_FACE ( 'NONE', ( #9783 ), #50548, .T. ) ;
#102638=CARTESIAN_POINT ( 'NONE',  ( 12.49999999999990230, 2.500000000000000000, -0.6928203230275541413 ) ) ;
#102639=CARTESIAN_POINT ( 'NONE',  ( 4.599999999999940137, 2.500000000000000000, -4.922947341949753586 ) ) ;
#102640=CONICAL_SURFACE ( 'NONE', #6466, 0.1000000000000000472, 0.003490658503988666988 ) ;
#102641=EDGE_CURVE ( 'NONE', #30880, #62242, #30742, .T. ) ;
#102642=CIRCLE ( 'NONE', #21172, 0.09999999999999982514 ) ;
#102643=EDGE_LOOP ( 'NONE', ( #55982, #489, #9127, #78668 ) ) ;
#102644=EDGE_CURVE ( 'NONE', #10609, #116681, #20898, .T. ) ;
#102645=DIRECTION ( 'NONE',  ( 0.000000000000000000, 0.000000000000000000, 1.000000000000000000 ) ) ;
#102646=ADVANCED_FACE ( 'NONE', ( #124259 ), #43144, .T. ) ;
#102647=FACE_OUTER_BOUND ( 'NONE', #114196, .T. ) ;
#102648=CARTESIAN_POINT ( 'NONE',  ( 2.499999999999948930, 2.500000000000000000, -5.022947341949754119 ) ) ;
#102649=EDGE_LOOP ( 'NONE', ( #78437, #37391, #123778, #23850 ) ) ;
#102650=CARTESIAN_POINT ( 'NONE',  ( -12.04999999999999716, 2.500000000000000000, -2.065063509461098068 ) ) ;
#102651=ADVANCED_FACE ( 'NONE', ( #22855 ), #115283, .T. ) ;
#102653=VECTOR ( 'NONE', #67893, 1000.000000000000000 ) ;
#102654=ORIENTED_EDGE ( 'NONE', *, *, #67633, .F. ) ;
#102655=AXIS2_PLACEMENT_3D ( 'NONE', #97856, #18654, #59901 ) ;
#102656=EDGE_LOOP ( 'NONE', ( #55999, #88841 ) ) ;
#102657=ORIENTED_EDGE ( 'NONE', *, *, #124902, .F. ) ;
#102658=ORIENTED_EDGE ( 'NONE', *, *, #43777, .T. ) ;
#102659=CARTESIAN_POINT ( 'NONE',  ( -14.79999999999998295, 12.50000000000000000, -0.4115034346978134749 ) ) ;
#102660=DIRECTION ( 'NONE',  ( -0.000000000000000000, 1.000000000000000000, -0.000000000000000000 ) ) ;
#102661=DIRECTION ( 'NONE',  ( 0.000000000000000000, 0.000000000000000000, -1.000000000000000000 ) ) ;
#102662=DIRECTION ( 'NONE',  ( 0.000000000000000000, 0.000000000000000000, -1.000000000000000000 ) ) ;
#102663=ORIENTED_EDGE ( 'NONE', *, *, #119492, .T. ) ;
#102664=AXIS2_PLACEMENT_3D ( 'NONE', #69060, #108967, #19308 ) ;
#102665=AXIS2_PLACEMENT_3D ( 'NONE', #65249, #105188, #15510 ) ;
#102666=CARTESIAN_POINT ( 'NONE',  ( -7.499999999999980460, 12.50000000000000000, -2.276824562219559311E-15 ) ) ;
#102667=ORIENTED_EDGE ( 'NONE', *, *, #49910, .T. ) ;
#102668=CARTESIAN_POINT ( 'NONE',  ( 3.099999999999943245, 2.500000000000000000, 4.083716857408420609 ) ) ;
#102669=CARTESIAN_POINT ( 'NONE',  ( -1.700000000000034817, 2.500000000000000000, -4.330127018922201643 ) ) ;
#102670=DIRECTION ( 'NONE',  ( 0.000000000000000000, 0.000000000000000000, -1.000000000000000000 ) ) ;
#102671=CARTESIAN_POINT ( 'NONE',  ( 9.799999999999913669, 12.50000000000000000, -3.918623584224389056 ) ) ;
#102672=EDGE_LOOP ( 'NONE', ( #51898, #76836, #27141, #84792 ) ) ;
#102673=VERTEX_POINT ( 'NONE', #51663 ) ;
#102674=EDGE_LOOP ( 'NONE', ( #4498, #108545 ) ) ;
#102675=DIRECTION ( 'NONE',  ( -0.000000000000000000, 1.000000000000000000, -0.000000000000000000 ) ) ;
#102676=DIRECTION ( 'NONE',  ( 0.000000000000000000, -0.9999939076577903929, 0.003490651415223739937 ) ) ;
#102677=CARTESIAN_POINT ( 'NONE',  ( 3.349999999999941913, 2.500000000000000000, 5.902370205355745192 ) ) ;
#102678=FACE_BOUND ( 'NONE', #67692, .T. ) ;
#102679=DIRECTION ( 'NONE',  ( 0.000000000000000000, 0.000000000000000000, 1.000000000000000000 ) ) ;
#102680=CARTESIAN_POINT ( 'NONE',  ( -13.74999999999998934, 2.500000000000000000, 2.957883832488652942 ) ) ;
#102681=CARTESIAN_POINT ( 'NONE',  ( -4.350000000000027178, 12.50000000000000000, -6.148780366869526226 ) ) ;
#102682=EDGE_CURVE ( 'NONE', #47303, #116756, #113796, .T. ) ;
#102683=AXIS2_PLACEMENT_3D ( 'NONE', #35340, #25492, #65426 ) ;
#102684=AXIS2_PLACEMENT_3D ( 'NONE', #108102, #117919, #18438 ) ;
#102685=DIRECTION ( 'NONE',  ( 0.000000000000000000, 1.000000000000000000, 0.000000000000000000 ) ) ;
#102686=VECTOR ( 'NONE', #93279, 1000.000000000000000 ) ;
#102688=CARTESIAN_POINT ( 'NONE',  ( 3.299999999999942979, 2.500000000000000000, 4.430127018922196847 ) ) ;
#102689=ORIENTED_EDGE ( 'NONE', *, *, #57739, .T. ) ;
#102690=DIRECTION ( 'NONE',  ( 0.000000000000000000, 0.000000000000000000, 1.000000000000000000 ) ) ;
#102691=AXIS2_PLACEMENT_3D ( 'NONE', #68452, #29836, #69753 ) ;
#102692=ORIENTED_EDGE ( 'NONE', *, *, #49902, .T. ) ;
#102693=EDGE_LOOP ( 'NONE', ( #90439, #82746 ) ) ;
#102694=CONICAL_SURFACE ( 'NONE', #46267, 0.09999999999999982514, 0.003490658503988666988 ) ;
#102695=DIRECTION ( 'NONE',  ( -0.000000000000000000, 1.000000000000000000, -0.000000000000000000 ) ) ;
#102696=EDGE_CURVE ( 'NONE', #55696, #49092, #44404, .T. ) ;
#102698=FACE_BOUND ( 'NONE', #79515, .T. ) ;
#102699=CARTESIAN_POINT ( 'NONE',  ( 11.64999999999990798, 2.500000000000000000, 5.702370205355745014 ) ) ;
#102700=EDGE_LOOP ( 'NONE', ( #76905, #41617 ) ) ;
#102702=CARTESIAN_POINT ( 'NONE',  ( -9.150000000000009237, 2.500000000000000000, 1.372243186433545370 ) ) ;
#102703=ORIENTED_EDGE ( 'NONE', *, *, #90955, .F. ) ;
#102704=DIRECTION ( 'NONE',  ( 0.000000000000000000, 0.000000000000000000, 1.000000000000000000 ) ) ;
#102705=DIRECTION ( 'NONE',  ( 0.000000000000000000, 0.000000000000000000, 1.000000000000000000 ) ) ;
#102706=ORIENTED_EDGE ( 'NONE', *, *, #53473, .T. ) ;
#102707=CARTESIAN_POINT ( 'NONE',  ( -0.6500000000000389910, 2.500000000000000000, -1.918653347947326004 ) ) ;
#102709=CIRCLE ( 'NONE', #77676, 0.06509327318403745899 ) ;
#102710=AXIS2_PLACEMENT_3D ( 'NONE', #103607, #121303, #23104 ) ;
#102712=ADVANCED_FACE ( 'NONE', ( #73225 ), #106979, .T. ) ;
#102713=DIRECTION ( 'NONE',  ( 0.000000000000000000, 1.000000000000000000, 0.000000000000000000 ) ) ;
#102714=DIRECTION ( 'NONE',  ( 0.000000000000000000, 0.000000000000000000, -1.000000000000000000 ) ) ;
#102715=LINE ( 'NONE', #53637, #53479 ) ;
#102716=ORIENTED_EDGE ( 'NONE', *, *, #110636, .F. ) ;
#102717=ORIENTED_EDGE ( 'NONE', *, *, #45706, .T. ) ;
#102719=AXIS2_PLACEMENT_3D ( 'NONE', #1259, #62125, #52297 ) ;
#102720=EDGE_CURVE ( 'NONE', #86983, #74378, #53591, .T. ) ;
#102721=ORIENTED_EDGE ( 'NONE', *, *, #39790, .F. ) ;
#102722=DIRECTION ( 'NONE',  ( -0.000000000000000000, -1.000000000000000000, -0.000000000000000000 ) ) ;
#102723=AXIS2_PLACEMENT_3D ( 'NONE', #71371, #83786, #123689 ) ;
#102725=ORIENTED_EDGE ( 'NONE', *, *, #57511, .T. ) ;
#102726=AXIS2_PLACEMENT_3D ( 'NONE', #48899, #37775, #18120 ) ;
#102727=CARTESIAN_POINT ( 'NONE',  ( -6.900000000000019007, 12.50000000000000000, -0.3464101615137783474 ) ) ;
#102728=DIRECTION ( 'NONE',  ( 0.000000000000000000, -0.9999939076577903929, 0.003490651415223739937 ) ) ;
#102730=EDGE_CURVE ( 'NONE', #20150, #113637, #32682, .T. ) ;
#102731=EDGE_CURVE ( 'NONE', #119576, #56267, #61486, .T. ) ;
#102732=CARTESIAN_POINT ( 'NONE',  ( -11.89999999999999680, 12.50000000000000000, -0.4115034346978116431 ) ) ;
#102733=ADVANCED_FACE ( 'NONE', ( #122971 ), #8676, .T. ) ;
#102734=EDGE_CURVE ( 'NONE', #129244, #128672, #63403, .T. ) ;
#102735=EDGE_CURVE ( 'NONE', #87361, #69532, #100629, .T. ) ;
#102736=DIRECTION ( 'NONE',  ( -0.000000000000000000, 1.000000000000000000, -0.000000000000000000 ) ) ;
#102737=AXIS2_PLACEMENT_3D ( 'NONE', #14275, #14896, #6365 ) ;
#102738=ORIENTED_EDGE ( 'NONE', *, *, #56602, .F. ) ;
#102739=VECTOR ( 'NONE', #7538, 1000.000000000000000 ) ;
#102740=ORIENTED_EDGE ( 'NONE', *, *, #60573, .F. ) ;
#102741=FACE_OUTER_BOUND ( 'NONE', #606, .T. ) ;
#102742=ORIENTED_EDGE ( 'NONE', *, *, #97187, .F. ) ;
#102744=CONICAL_SURFACE ( 'NONE', #23322, 0.1000000000000002554, 0.003490658503988666988 ) ;
#102745=ORIENTED_EDGE ( 'NONE', *, *, #86352, .F. ) ;
#102746=ORIENTED_EDGE ( 'NONE', *, *, #74408, .F. ) ;
#102747=ORIENTED_EDGE ( 'NONE', *, *, #40293, .F. ) ;
#102748=ADVANCED_FACE ( 'NONE', ( #1893 ), #19141, .T. ) ;
#102749=CARTESIAN_POINT ( 'NONE',  ( 0.6499999999999566125, 2.500000000000000000, -6.841600689897077814 ) ) ;
#102750=AXIS2_PLACEMENT_3D ( 'NONE', #21902, #70340, #101739 ) ;
#102751=EDGE_CURVE ( 'NONE', #95146, #17807, #103975, .T. ) ;
#102752=CARTESIAN_POINT ( 'NONE',  ( -12.49999999999995737, 12.50000000000000000, 4.330127018922196314 ) ) ;
#102753=ADVANCED_FACE ( 'NONE', ( #24126 ), #88095, .T. ) ;
#102754=CARTESIAN_POINT ( 'NONE',  ( -7.100000000000018296, 12.50000000000000000, -4.330127018922201643 ) ) ;
#102755=CARTESIAN_POINT ( 'NONE',  ( -5.400000000000024336, 2.500000000000000000, -3.637306695894650055 ) ) ;
#102756=VECTOR ( 'NONE', #1670, 1000.000000000000000 ) ;
#102757=DIRECTION ( 'NONE',  ( 0.000000000000000000, 0.000000000000000000, 1.000000000000000000 ) ) ;
#102758=DIRECTION ( 'NONE',  ( 0.000000000000000000, 1.000000000000000000, 0.000000000000000000 ) ) ;
#102759=DIRECTION ( 'NONE',  ( 0.000000000000000000, -0.000000000000000000, 1.000000000000000000 ) ) ;
#102760=DIRECTION ( 'NONE',  ( 0.000000000000000000, 0.000000000000000000, -1.000000000000000000 ) ) ;
#102761=CARTESIAN_POINT ( 'NONE',  ( -11.84999999999999609, 12.50000000000000000, 1.753560074763284016 ) ) ;
#102762=VERTEX_POINT ( 'NONE', #84324 ) ;
#102763=DIRECTION ( 'NONE',  ( 0.000000000000000000, 0.000000000000000000, -1.000000000000000000 ) ) ;
#102764=ORIENTED_EDGE ( 'NONE', *, *, #77296, .T. ) ;
#102765=ORIENTED_EDGE ( 'NONE', *, *, #91527, .F. ) ;
#102766=CARTESIAN_POINT ( 'NONE',  ( -2.050000000000033129, 2.500000000000000000, 6.595190528383296780 ) ) ;
#102767=CARTESIAN_POINT ( 'NONE',  ( 11.04999999999990656, 2.500000000000000000, 2.411473670974873862 ) ) ;
#102768=CARTESIAN_POINT ( 'NONE',  ( -7.300000000000016698, 12.50000000000000000, -0.3464101615137783474 ) ) ;
#102769=FACE_OUTER_BOUND ( 'NONE', #7924, .T. ) ;
#102770=CARTESIAN_POINT ( 'NONE',  ( 12.29999999999990656, 2.500000000000000000, 3.983716857408420964 ) ) ;
#102771=DIRECTION ( 'NONE',  ( 0.000000000000000000, 0.000000000000000000, 1.000000000000000000 ) ) ;
#102772=DIRECTION ( 'NONE',  ( 0.000000000000000000, 0.000000000000000000, 1.000000000000000000 ) ) ;
#102773=EDGE_LOOP ( 'NONE', ( #50608, #27249, #26006, #59666 ) ) ;
#102774=VECTOR ( 'NONE', #1057, 1000.000000000000000 ) ;
#102775=AXIS2_PLACEMENT_3D ( 'NONE', #11979, #70268, #31634 ) ;
#102776=EDGE_LOOP ( 'NONE', ( #40458, #23780 ) ) ;
#102777=CONICAL_SURFACE ( 'NONE', #27463, 0.09999999999999982514, 0.003490658503988666988 ) ;
#102778=ORIENTED_EDGE ( 'NONE', *, *, #75489, .F. ) ;
#102779=CONICAL_SURFACE ( 'NONE', #77733, 0.09999999999999999167, 0.003490658503988666988 ) ;
#102780=ORIENTED_EDGE ( 'NONE', *, *, #14820, .F. ) ;
#102781=CONICAL_SURFACE ( 'NONE', #48416, 0.1000000000000002554, 0.003490658503988666988 ) ;
#102782=AXIS2_PLACEMENT_3D ( 'NONE', #23798, #2198, #121996 ) ;
#102783=EDGE_CURVE ( 'NONE', #31905, #60176, #81851, .T. ) ;
#102784=VERTEX_POINT ( 'NONE', #33945 ) ;
#102785=DIRECTION ( 'NONE',  ( 0.000000000000000000, -0.9999939076577903929, 0.003490651415223739937 ) ) ;
#102786=DIRECTION ( 'NONE',  ( -4.274815082592931898E-19, -0.9999939076577903929, -0.003490651415223739937 ) ) ;
#102788=EDGE_CURVE ( 'NONE', #127817, #120673, #98566, .T. ) ;
#102789=LINE ( 'NONE', #3954, #69633 ) ;
#102790=DIRECTION ( 'NONE',  ( 0.000000000000000000, 0.000000000000000000, 1.000000000000000000 ) ) ;
#102791=EDGE_CURVE ( 'NONE', #127159, #104514, #83912, .T. ) ;
#102792=LINE ( 'NONE', #84461, #86893 ) ;
#102793=ORIENTED_EDGE ( 'NONE', *, *, #95531, .F. ) ;
#102794=CARTESIAN_POINT ( 'NONE',  ( 21.24754738303277080, -0.7337760880902354232, 4.182111650399362723 ) ) ;
#102795=CARTESIAN_POINT ( 'NONE',  ( 1.649999999999949729, 2.500000000000000000, 5.902370205355745192 ) ) ;
#102796=DIRECTION ( 'NONE',  ( 0.000000000000000000, 0.000000000000000000, 1.000000000000000000 ) ) ;
#102797=ADVANCED_FACE ( 'NONE', ( #72586 ), #27318, .T. ) ;
#102798=DIRECTION ( 'NONE',  ( 0.000000000000000000, 1.000000000000000000, 0.000000000000000000 ) ) ;
#102799=ORIENTED_EDGE ( 'NONE', *, *, #28127, .T. ) ;
#102800=VERTEX_POINT ( 'NONE', #105253 ) ;
#102802=DIRECTION ( 'NONE',  ( 0.000000000000000000, 0.000000000000000000, -1.000000000000000000 ) ) ;
#102803=EDGE_CURVE ( 'NONE', #93446, #69877, #96709, .T. ) ;
#102804=DIRECTION ( 'NONE',  ( -4.274815082592931898E-19, -0.9999939076577903929, -0.003490651415223739937 ) ) ;
#102806=LINE ( 'NONE', #43281, #106673 ) ;
#102807=AXIS2_PLACEMENT_3D ( 'NONE', #2164, #92482, #44039 ) ;
#102808=ORIENTED_EDGE ( 'NONE', *, *, #64687, .T. ) ;
#102809=CARTESIAN_POINT ( 'NONE',  ( 14.14999999999989200, 2.500000000000000000, -2.065063509461102065 ) ) ;
#102810=DIRECTION ( 'NONE',  ( 0.000000000000000000, 0.000000000000000000, -1.000000000000000000 ) ) ;
#102811=DIRECTION ( 'NONE',  ( 0.000000000000000000, 0.000000000000000000, -1.000000000000000000 ) ) ;
#102812=EDGE_CURVE ( 'NONE', #5452, #64674, #29631, .T. ) ;
#102813=DIRECTION ( 'NONE',  ( -0.000000000000000000, 1.000000000000000000, -0.000000000000000000 ) ) ;
#102814=CIRCLE ( 'NONE', #113287, 0.06509327318403745899 ) ;
#102815=VECTOR ( 'NONE', #15333, 1000.000000000000000 ) ;
#102816=VECTOR ( 'NONE', #66246, 1000.000000000000000 ) ;
#102817=CARTESIAN_POINT ( 'NONE',  ( 5.399999999999935518, 2.500000000000000000, -4.330127018922201643 ) ) ;
#102818=ORIENTED_EDGE ( 'NONE', *, *, #119379, .F. ) ;
#102819=ORIENTED_EDGE ( 'NONE', *, *, #15628, .T. ) ;
#102820=DIRECTION ( 'NONE',  ( 0.000000000000000000, 0.000000000000000000, 1.000000000000000000 ) ) ;
#102821=CARTESIAN_POINT ( 'NONE',  ( -9.600000000000006750, 12.50000000000000000, 3.637306695894644726 ) ) ;
#102822=DIRECTION ( 'NONE',  ( 0.000000000000000000, 0.000000000000000000, -1.000000000000000000 ) ) ;
#102823=AXIS2_PLACEMENT_3D ( 'NONE', #68381, #9473, #27173 ) ;
#102824=AXIS2_PLACEMENT_3D ( 'NONE', #91268, #122023, #71624 ) ;
#102825=DIRECTION ( 'NONE',  ( 0.000000000000000000, 0.000000000000000000, 1.000000000000000000 ) ) ;
#102826=ORIENTED_EDGE ( 'NONE', *, *, #59533, .F. ) ;
#102827=ADVANCED_FACE ( 'NONE', ( #6374 ), #102777, .T. ) ;
#102828=AXIS2_PLACEMENT_3D ( 'NONE', #127816, #21081, #20450 ) ;
#102829=AXIS2_PLACEMENT_3D ( 'NONE', #56403, #128401, #116611 ) ;
#102830=CIRCLE ( 'NONE', #88151, 0.06509327318403745899 ) ;
#102831=ORIENTED_EDGE ( 'NONE', *, *, #128228, .T. ) ;
#102832=FACE_OUTER_BOUND ( 'NONE', #41746, .T. ) ;
#102833=CARTESIAN_POINT ( 'NONE',  ( 3.349999999999941913, 2.500000000000000000, 6.595190528383296780 ) ) ;
#102834=CIRCLE ( 'NONE', #117486, 0.06509327318403741736 ) ;
#102835=DIRECTION ( 'NONE',  ( -0.000000000000000000, 1.000000000000000000, -0.000000000000000000 ) ) ;
#102837=ORIENTED_EDGE ( 'NONE', *, *, #54823, .T. ) ;
#102838=CARTESIAN_POINT ( 'NONE',  ( -10.65000000000000391, 2.500000000000000000, -2.511473670974873951 ) ) ;
#102839=CARTESIAN_POINT ( 'NONE',  ( 3.299999999999944755, 2.500000000000000000, 0.09999999999999761857 ) ) ;
#102840=CIRCLE ( 'NONE', #63148, 0.06509327318403745899 ) ;
#102841=EDGE_LOOP ( 'NONE', ( #23206, #66200 ) ) ;
#102842=DIRECTION ( 'NONE',  ( -0.000000000000000000, 1.000000000000000000, -0.000000000000000000 ) ) ;
#102843=EDGE_CURVE ( 'NONE', #48868, #90822, #119511, .T. ) ;
#102844=VERTEX_POINT ( 'NONE', #77088 ) ;
#102845=B_SPLINE_CURVE_WITH_KNOTS ( 'NONE', 3,
 ( #82034, #71575, #72874, #121977, #82708, #112157 ),
 .UNSPECIFIED., .F., .F.,
 ( 4, 2, 4 ),
 ( 0.000000000000000000, 0.5000000000000000000, 1.000000000000000000 ),
 .UNSPECIFIED. ) ;
#102846=DIRECTION ( 'NONE',  ( 0.000000000000000000, 0.000000000000000000, 1.000000000000000000 ) ) ;
#102847=VERTEX_POINT ( 'NONE', #116987 ) ;
#102848=DIRECTION ( 'NONE',  ( 0.000000000000000000, 1.000000000000000000, 0.000000000000000000 ) ) ;
#102849=LINE ( 'NONE', #13174, #25102 ) ;
#102850=VERTEX_POINT ( 'NONE', #87538 ) ;
#102851=ADVANCED_FACE ( 'NONE', ( #55520 ), #58981, .T. ) ;
#102852=ORIENTED_EDGE ( 'NONE', *, *, #21665, .T. ) ;
#102856=PLANE ( 'NONE',  #30449 ) ;
#102857=CARTESIAN_POINT ( 'NONE',  ( 4.999999999999938716, 12.50000000000000000, -5.022947341949754119 ) ) ;
#102858=CARTESIAN_POINT ( 'NONE',  ( -4.150000000000024336, 2.500000000000000000, -2.265063509461101798 ) ) ;
#102859=DIRECTION ( 'NONE',  ( 0.000000000000000000, 0.000000000000000000, -1.000000000000000000 ) ) ;
#102861=CONICAL_SURFACE ( 'NONE', #42254, 0.1000000000000002554, 0.003490658503988666988 ) ;
#102862=DIRECTION ( 'NONE',  ( -4.274815082592931898E-19, -0.9999939076577903929, -0.003490651415223739937 ) ) ;
#102863=LINE ( 'NONE', #3389, #12852 ) ;
#102864=CIRCLE ( 'NONE', #73627, 0.09999999999999982514 ) ;
#102865=VERTEX_POINT ( 'NONE', #16837 ) ;
#102866=AXIS2_PLACEMENT_3D ( 'NONE', #22925, #33400, #62215 ) ;
#102867=ADVANCED_FACE ( 'NONE', ( #5742 ), #107075, .T. ) ;
#102868=VERTEX_POINT ( 'NONE', #57449 ) ;
#102870=ORIENTED_EDGE ( 'NONE', *, *, #86744, .T. ) ;
#102871=CARTESIAN_POINT ( 'NONE',  ( 0.3999999999999628852, 2.500000000000000000, 0.5928203230275517210 ) ) ;
#102872=CARTESIAN_POINT ( 'NONE',  ( 4.349999999999938360, 2.500000000000000000, 1.918653347947321564 ) ) ;
#102873=AXIS2_PLACEMENT_3D ( 'NONE', #56534, #96451, #46731 ) ;
#102874=DIRECTION ( 'NONE',  ( -0.000000000000000000, 1.000000000000000000, -0.000000000000000000 ) ) ;
#102876=ORIENTED_EDGE ( 'NONE', *, *, #26912, .T. ) ;
#102877=VERTEX_POINT ( 'NONE', #45704 ) ;
#102878=FACE_BOUND ( 'NONE', #23143, .T. ) ;
#102879=ORIENTED_EDGE ( 'NONE', *, *, #5676, .T. ) ;
#102880=FACE_OUTER_BOUND ( 'NONE', #41115, .T. ) ;
#102881=DIRECTION ( 'NONE',  ( -0.000000000000000000, -1.000000000000000000, -0.000000000000000000 ) ) ;
#102882=AXIS2_PLACEMENT_3D ( 'NONE', #5068, #96034, #116303 ) ;
#102883=DIRECTION ( 'NONE',  ( 0.000000000000000000, 0.000000000000000000, -1.000000000000000000 ) ) ;
#102885=DIRECTION ( 'NONE',  ( -0.000000000000000000, 1.000000000000000000, -0.000000000000000000 ) ) ;
#102887=DIRECTION ( 'NONE',  ( -0.000000000000000000, -1.000000000000000000, -0.000000000000000000 ) ) ;
#102888=CARTESIAN_POINT ( 'NONE',  ( -3.749999999999991562, 12.50000000000000000, 6.560283801567334372 ) ) ;
#102889=CARTESIAN_POINT ( 'NONE',  ( -0.6500000000000398792, 2.500000000000000000, -2.511473670974877948 ) ) ;
#102890=ADVANCED_FACE ( 'NONE', ( #56143 ), #15026, .T. ) ;
#102891=ADVANCED_FACE ( 'NONE', ( #126833 ), #61019, .T. ) ;
#102892=DIRECTION ( 'NONE',  ( -0.000000000000000000, -1.000000000000000000, -0.000000000000000000 ) ) ;
#102893=DIRECTION ( 'NONE',  ( -4.274815082592931898E-19, -0.9999939076577903929, -0.003490651415223739937 ) ) ;
#102894=ADVANCED_FACE ( 'NONE', ( #36536 ), #84966, .T. ) ;
#102896=DIRECTION ( 'NONE',  ( -0.000000000000000000, -1.000000000000000000, -0.000000000000000000 ) ) ;
#102897=ORIENTED_EDGE ( 'NONE', *, *, #38518, .F. ) ;
#102898=VERTEX_POINT ( 'NONE', #65316 ) ;
#102899=ORIENTED_EDGE ( 'NONE', *, *, #51542, .T. ) ;
#102900=DIRECTION ( 'NONE',  ( -0.000000000000000000, -1.000000000000000000, -0.000000000000000000 ) ) ;
#102901=ORIENTED_EDGE ( 'NONE', *, *, #129538, .T. ) ;
#102902=EDGE_CURVE ( 'NONE', #100484, #72434, #86897, .T. ) ;
#102903=FACE_OUTER_BOUND ( 'NONE', #26175, .T. ) ;
#102904=EDGE_CURVE ( 'NONE', #41615, #125433, #115708, .T. ) ;
#102905=ORIENTED_EDGE ( 'NONE', *, *, #97709, .T. ) ;
#102906=EDGE_LOOP ( 'NONE', ( #5902, #93405 ) ) ;
#102907=ORIENTED_EDGE ( 'NONE', *, *, #5228, .F. ) ;
#102908=ADVANCED_FACE ( 'NONE', ( #65975 ), #48512, .T. ) ;
#102909=DIRECTION ( 'NONE',  ( -0.000000000000000000, -1.000000000000000000, -0.000000000000000000 ) ) ;
#102910=CIRCLE ( 'NONE', #42378, 0.06509327318403741736 ) ;
#102911=ADVANCED_FACE ( 'NONE', ( #69177 ), #29727, .T. ) ;
#102912=EDGE_CURVE ( 'NONE', #108868, #38667, #102864, .T. ) ;
#102913=DIRECTION ( 'NONE',  ( -0.000000000000000000, 1.000000000000000000, -0.000000000000000000 ) ) ;
#102914=CARTESIAN_POINT ( 'NONE',  ( -11.04999999999999893, 12.50000000000000000, 6.213873640053558134 ) ) ;
#102915=DIRECTION ( 'NONE',  ( 0.000000000000000000, 0.000000000000000000, 1.000000000000000000 ) ) ;
#102916=DIRECTION ( 'NONE',  ( 0.000000000000000000, -0.000000000000000000, 1.000000000000000000 ) ) ;
#102917=ORIENTED_EDGE ( 'NONE', *, *, #59039, .F. ) ;
#102918=VECTOR ( 'NONE', #93993, 1000.000000000000000 ) ;
#102919=ADVANCED_FACE ( 'NONE', ( #102372 ), #112122, .T. ) ;
#102921=DIRECTION ( 'NONE',  ( 0.000000000000000000, -0.000000000000000000, 1.000000000000000000 ) ) ;
#102922=EDGE_LOOP ( 'NONE', ( #21411, #18934, #50430, #101267 ) ) ;
#102923=CIRCLE ( 'NONE', #25649, 0.09999999999999982514 ) ;
#102924=ORIENTED_EDGE ( 'NONE', *, *, #77597, .T. ) ;
#102925=CIRCLE ( 'NONE', #44437, 0.06509327318403745899 ) ;
#102926=ORIENTED_EDGE ( 'NONE', *, *, #41608, .F. ) ;
#102927=DIRECTION ( 'NONE',  ( 0.000000000000000000, 1.000000000000000000, 0.000000000000000000 ) ) ;
#102929=VERTEX_POINT ( 'NONE', #39124 ) ;
#102930=ORIENTED_EDGE ( 'NONE', *, *, #64061, .F. ) ;
#102931=EDGE_LOOP ( 'NONE', ( #70991, #35119 ) ) ;
#102932=AXIS2_PLACEMENT_3D ( 'NONE', #23635, #60529, #93031 ) ;
#102933=DIRECTION ( 'NONE',  ( 0.000000000000000000, -0.000000000000000000, 1.000000000000000000 ) ) ;
#102934=AXIS2_PLACEMENT_3D ( 'NONE', #53130, #102848, #43320 ) ;
#102935=CARTESIAN_POINT ( 'NONE',  ( -8.749999999999975131, 2.500000000000000000, 2.165063509461097713 ) ) ;
#102936=CARTESIAN_POINT ( 'NONE',  ( 13.29999999999990301, 2.500000000000000000, -4.330127018922201643 ) ) ;
#102937=CARTESIAN_POINT ( 'NONE',  ( 5.199999999999931788, 12.50000000000000000, 4.676537180435972552 ) ) ;
#102938=AXIS2_PLACEMENT_3D ( 'NONE', #31463, #52382, #64129 ) ;
#102939=DIRECTION ( 'NONE',  ( 0.000000000000000000, 0.000000000000000000, 1.000000000000000000 ) ) ;
#102940=AXIS2_PLACEMENT_3D ( 'NONE', #58365, #88437, #38737 ) ;
#102941=CIRCLE ( 'NONE', #109188, 0.09999999999999982514 ) ;
#102942=CARTESIAN_POINT ( 'NONE',  ( -4.350000000000027178, 2.500000000000000000, -6.941600689897077459 ) ) ;
#102943=VECTOR ( 'NONE', #13010, 1000.000000000000000 ) ;
#102944=DIRECTION ( 'NONE',  ( 0.000000000000000000, 1.000000000000000000, 0.000000000000000000 ) ) ;
#102945=ORIENTED_EDGE ( 'NONE', *, *, #128472, .T. ) ;
#102946=PLANE ( 'NONE',  #121596 ) ;
#102947=ORIENTED_EDGE ( 'NONE', *, *, #49919, .F. ) ;
#102948=CARTESIAN_POINT ( 'NONE',  ( 4.399999999999939071, 12.50000000000000000, 0.4115034346978110880 ) ) ;
#102949=VERTEX_POINT ( 'NONE', #22538 ) ;
#102950=VERTEX_POINT ( 'NONE', #51988 ) ;
#102952=ADVANCED_FACE ( 'NONE', ( #78390 ), #10910, .T. ) ;
#102953=DIRECTION ( 'NONE',  ( 0.000000000000000000, 0.000000000000000000, 1.000000000000000000 ) ) ;
#102954=EDGE_CURVE ( 'NONE', #1645, #124183, #2515, .T. ) ;
#102955=VERTEX_POINT ( 'NONE', #77711 ) ;
#102956=ORIENTED_EDGE ( 'NONE', *, *, #14254, .F. ) ;
#102957=DIRECTION ( 'NONE',  ( -0.000000000000000000, 1.000000000000000000, -0.000000000000000000 ) ) ;
#102958=DIRECTION ( 'NONE',  ( 0.000000000000000000, 1.000000000000000000, 0.000000000000000000 ) ) ;
#102959=AXIS2_PLACEMENT_3D ( 'NONE', #32154, #81862, #52413 ) ;
#102960=CARTESIAN_POINT ( 'NONE',  ( -5.000000000000026645, 12.50000000000000000, -3.572213422710612374 ) ) ;
#102961=CARTESIAN_POINT ( 'NONE',  ( -11.24999999999996270, 2.500000000000000000, 6.495190528383297135 ) ) ;
#102962=ADVANCED_FACE ( 'NONE', ( #108468 ), #54752, .T. ) ;
#102963=LINE ( 'NONE', #113435, #68736 ) ;
#102964=ORIENTED_EDGE ( 'NONE', *, *, #102904, .F. ) ;
#102965=DIRECTION ( 'NONE',  ( 1.000000000000000000, -0.000000000000000000, -0.000000000000000000 ) ) ;
#102966=CONICAL_SURFACE ( 'NONE', #61211, 0.1000000000000002554, 0.003490658503988666988 ) ;
#102967=VECTOR ( 'NONE', #71338, 1000.000000000000000 ) ;
#102968=AXIS2_PLACEMENT_3D ( 'NONE', #57566, #106650, #96822 ) ;
#102969=ORIENTED_EDGE ( 'NONE', *, *, #12703, .T. ) ;
#102971=DIRECTION ( 'NONE',  ( 0.000000000000000000, 0.000000000000000000, -1.000000000000000000 ) ) ;
#102972=CIRCLE ( 'NONE', #50754, 0.06509327318403745899 ) ;
#102973=AXIS2_PLACEMENT_3D ( 'NONE', #14260, #122309, #43121 ) ;
#102974=AXIS2_PLACEMENT_3D ( 'NONE', #5557, #36972, #65770 ) ;
#102975=VECTOR ( 'NONE', #7110, 1000.000000000000000 ) ;
#102976=VECTOR ( 'NONE', #19298, 1000.000000000000000 ) ;
#102978=DIRECTION ( 'NONE',  ( -0.000000000000000000, 1.000000000000000000, -0.000000000000000000 ) ) ;
#102979=CARTESIAN_POINT ( 'NONE',  ( -7.100000000000017408, 12.50000000000000000, -5.022947341949754119 ) ) ;
#102980=DIRECTION ( 'NONE',  ( 0.000000000000000000, 0.000000000000000000, -1.000000000000000000 ) ) ;
#102982=ORIENTED_EDGE ( 'NONE', *, *, #80140, .F. ) ;
#102983=DIRECTION ( 'NONE',  ( 0.000000000000000000, 1.000000000000000000, 0.000000000000000000 ) ) ;
#102984=FACE_OUTER_BOUND ( 'NONE', #6781, .T. ) ;
#102985=DIRECTION ( 'NONE',  ( 0.000000000000000000, 0.000000000000000000, 1.000000000000000000 ) ) ;
#102986=ORIENTED_EDGE ( 'NONE', *, *, #75973, .F. ) ;
#102987=CARTESIAN_POINT ( 'NONE',  ( -7.300000000000016698, 12.50000000000000000, -4.676537180435978769 ) ) ;
#102988=AXIS2_PLACEMENT_3D ( 'NONE', #15241, #62455, #13965 ) ;
#102989=EDGE_CURVE ( 'NONE', #46118, #54643, #71479, .T. ) ;
#102990=EDGE_LOOP ( 'NONE', ( #52277, #82824, #53900, #65069 ) ) ;
#102991=EDGE_LOOP ( 'NONE', ( #31514, #8411, #9467, #25626 ) ) ;
#102992=DIRECTION ( 'NONE',  ( -0.000000000000000000, -1.000000000000000000, -0.000000000000000000 ) ) ;
#102993=EDGE_LOOP ( 'NONE', ( #85796, #32322 ) ) ;
#102994=CARTESIAN_POINT ( 'NONE',  ( 16.09541403887941158, -2.463474929527615487, -3.723514363715260789 ) ) ;
#102995=CARTESIAN_POINT ( 'NONE',  ( 11.44999999999990870, 2.500000000000000000, -1.818653347947326138 ) ) ;
#102996=DIRECTION ( 'NONE',  ( 0.000000000000000000, 0.000000000000000000, -1.000000000000000000 ) ) ;
#102997=CIRCLE ( 'NONE', #107204, 0.1000000000000000056 ) ;
#102998=ORIENTED_EDGE ( 'NONE', *, *, #120349, .T. ) ;
#102999=AXIS2_PLACEMENT_3D ( 'NONE', #47498, #39637, #99825 ) ;
#103000=CIRCLE ( 'NONE', #46565, 0.1000000000000000472 ) ;
#103001=FACE_OUTER_BOUND ( 'NONE', #79637, .T. ) ;
#103002=CARTESIAN_POINT ( 'NONE',  ( -5.650000000000023448, 2.500000000000000000, -1.718653347947326049 ) ) ;
#103004=EDGE_CURVE ( 'NONE', #92191, #74205, #4137, .T. ) ;
#103005=AXIS2_PLACEMENT_3D ( 'NONE', #17004, #97533, #56950 ) ;
#103006=ORIENTED_EDGE ( 'NONE', *, *, #79398, .F. ) ;
#103007=AXIS2_PLACEMENT_3D ( 'NONE', #55768, #29389, #90206 ) ;
#103008=AXIS2_PLACEMENT_3D ( 'NONE', #85824, #125739, #127063 ) ;
#103009=ORIENTED_EDGE ( 'NONE', *, *, #19844, .F. ) ;
#103010=VERTEX_POINT ( 'NONE', #63082 ) ;
#103011=CARTESIAN_POINT ( 'NONE',  ( -6.050000000000018474, 12.50000000000000000, 6.841600689897072485 ) ) ;
#103012=PLANE ( 'NONE',  #129514 ) ;
#103014=ADVANCED_FACE ( 'NONE', ( #5437 ), #33934, .T. ) ;
#103015=EDGE_LOOP ( 'NONE', ( #64844, #102027 ) ) ;
#103016=DIRECTION ( 'NONE',  ( 0.000000000000000000, 0.000000000000000000, -1.000000000000000000 ) ) ;
#103017=CARTESIAN_POINT ( 'NONE',  ( -1.650000000000034772, 12.50000000000000000, 1.472243186433545459 ) ) ;
#103018=ORIENTED_EDGE ( 'NONE', *, *, #41068, .F. ) ;
#103019=CONICAL_SURFACE ( 'NONE', #80047, 0.09999999999999982514, 0.003490658503988666988 ) ;
#103020=CARTESIAN_POINT ( 'NONE',  ( 2.499999999999947153, 12.50000000000000000, 0.7579135962115869374 ) ) ;
#103021=DIRECTION ( 'NONE',  ( 0.000000000000000000, 1.000000000000000000, 0.000000000000000000 ) ) ;
#103022=AXIS2_PLACEMENT_3D ( 'NONE', #33255, #12291, #73162 ) ;
#103023=AXIS2_PLACEMENT_3D ( 'NONE', #43853, #124327, #125593 ) ;
#103024=DIRECTION ( 'NONE',  ( 0.000000000000000000, 1.000000000000000000, 0.000000000000000000 ) ) ;
#103026=LINE ( 'NONE', #121378, #117646 ) ;
#103027=DIRECTION ( 'NONE',  ( -0.000000000000000000, -1.000000000000000000, -0.000000000000000000 ) ) ;
#103028=VECTOR ( 'NONE', #39155, 1000.000000000000000 ) ;
#103029=CARTESIAN_POINT ( 'NONE',  ( 6.249999999999934275, 12.50000000000000000, -7.253104124594891289 ) ) ;
#103030=EDGE_LOOP ( 'NONE', ( #94547, #44646, #107048, #24926 ) ) ;
#103031=CIRCLE ( 'NONE', #23620, 0.06509327318403745899 ) ;
#103032=ORIENTED_EDGE ( 'NONE', *, *, #65670, .T. ) ;
#103033=ORIENTED_EDGE ( 'NONE', *, *, #66101, .F. ) ;
#103034=EDGE_LOOP ( 'NONE', ( #53023, #91002 ) ) ;
#103035=CARTESIAN_POINT ( 'NONE',  ( -3.100000000000028511, 2.500000000000000000, -0.4464101615137782142 ) ) ;
#103036=CARTESIAN_POINT ( 'NONE',  ( -0.4000000000000396572, 2.500000000000000000, 3.737306695894644371 ) ) ;
#103037=CARTESIAN_POINT ( 'NONE',  ( 6.649999999999930189, 2.500000000000000000, -1.572243186433550211 ) ) ;
#103038=ORIENTED_EDGE ( 'NONE', *, *, #119478, .F. ) ;
#103039=FACE_BOUND ( 'NONE', #42105, .T. ) ;
#103040=DIRECTION ( 'NONE',  ( 0.000000000000000000, 0.000000000000000000, -1.000000000000000000 ) ) ;
#103041=CARTESIAN_POINT ( 'NONE',  ( -10.45000000000000107, 2.500000000000000000, 6.495190528383297135 ) ) ;
#103042=DIRECTION ( 'NONE',  ( 0.000000000000000000, 0.000000000000000000, 1.000000000000000000 ) ) ;
#103043=ADVANCED_FACE ( 'NONE', ( #73532 ), #104919, .T. ) ;
#103044=DIRECTION ( 'NONE',  ( -0.000000000000000000, -1.000000000000000000, -0.000000000000000000 ) ) ;
#103045=CARTESIAN_POINT ( 'NONE',  ( -6.250000000000021316, 12.50000000000000000, -1.537336459617587581 ) ) ;
#103046=DIRECTION ( 'NONE',  ( 0.000000000000000000, 0.000000000000000000, 1.000000000000000000 ) ) ;
#103047=DIRECTION ( 'NONE',  ( 0.000000000000000000, -0.9999939076577903929, 0.003490651415223739937 ) ) ;
#103048=CARTESIAN_POINT ( 'NONE',  ( 10.39999999999990976, 2.500000000000000000, -4.330127018922201643 ) ) ;
#103049=CONICAL_SURFACE ( 'NONE', #76156, 0.1000000000000002554, 0.003490658503988666988 ) ;
#103050=AXIS2_PLACEMENT_3D ( 'NONE', #126966, #117116, #98135 ) ;
#103051=ADVANCED_FACE ( 'NONE', ( #113466 ), #81941, .T. ) ;
#103052=DIRECTION ( 'NONE',  ( 0.000000000000000000, 0.000000000000000000, 1.000000000000000000 ) ) ;
#103053=EDGE_CURVE ( 'NONE', #1029, #82577, #63177, .T. ) ;
#103054=ORIENTED_EDGE ( 'NONE', *, *, #25571, .T. ) ;
#103055=CIRCLE ( 'NONE', #46624, 0.1000000000000002554 ) ;
#103056=ORIENTED_EDGE ( 'NONE', *, *, #43821, .F. ) ;
#103057=ORIENTED_EDGE ( 'NONE', *, *, #125513, .T. ) ;
#103058=EDGE_LOOP ( 'NONE', ( #55851, #68260, #117234, #70861 ) ) ;
#103059=AXIS2_PLACEMENT_3D ( 'NONE', #49776, #90968, #101431 ) ;
#103060=ORIENTED_EDGE ( 'NONE', *, *, #41554, .T. ) ;
#103061=CIRCLE ( 'NONE', #40487, 0.1000000000000002554 ) ;
#103062=EDGE_CURVE ( 'NONE', #69482, #16861, #25506, .T. ) ;
#103063=ORIENTED_EDGE ( 'NONE', *, *, #20464, .F. ) ;
#103064=CIRCLE ( 'NONE', #52902, 0.06509327318403745899 ) ;
#103065=DIRECTION ( 'NONE',  ( 0.000000000000000000, 1.000000000000000000, 0.000000000000000000 ) ) ;
#103066=EDGE_CURVE ( 'NONE', #24243, #83715, #12977, .T. ) ;
#103067=EDGE_CURVE ( 'NONE', #54959, #72089, #42258, .T. ) ;
#103068=ORIENTED_EDGE ( 'NONE', *, *, #19381, .F. ) ;
#103069=ORIENTED_EDGE ( 'NONE', *, *, #53001, .T. ) ;
#103070=AXIS2_PLACEMENT_3D ( 'NONE', #79143, #119057, #69285 ) ;
#103071=CIRCLE ( 'NONE', #82149, 0.09999999999999982514 ) ;
#103072=CIRCLE ( 'NONE', #44585, 0.09999999999999982514 ) ;
#103073=EDGE_CURVE ( 'NONE', #122978, #117692, #75680, .T. ) ;
#103074=CARTESIAN_POINT ( 'NONE',  ( 13.34999999999989662, 2.500000000000000000, -2.857883832488653741 ) ) ;
#103075=CARTESIAN_POINT ( 'NONE',  ( 5.399999999999931966, 2.500000000000000000, 4.330127018922196314 ) ) ;
#103076=DIRECTION ( 'NONE',  ( 0.000000000000000000, -0.9999939076577903929, 0.003490651415223739937 ) ) ;
#103077=AXIS2_PLACEMENT_3D ( 'NONE', #79735, #127549, #37874 ) ;
#103078=AXIS2_PLACEMENT_3D ( 'NONE', #11651, #12916, #32617 ) ;
#103079=VERTEX_POINT ( 'NONE', #104299 ) ;
#103080=DIRECTION ( 'NONE',  ( -0.000000000000000000, 1.000000000000000000, -0.000000000000000000 ) ) ;
#103081=EDGE_CURVE ( 'NONE', #62968, #50779, #44297, .T. ) ;
#103083=ORIENTED_EDGE ( 'NONE', *, *, #19427, .T. ) ;
#103084=VERTEX_POINT ( 'NONE', #44745 ) ;
#103085=DIRECTION ( 'NONE',  ( 0.000000000000000000, 0.000000000000000000, 1.000000000000000000 ) ) ;
#103086=CARTESIAN_POINT ( 'NONE',  ( -5.850000000000021849, 2.500000000000000000, -5.702370205355749455 ) ) ;
#103087=EDGE_LOOP ( 'NONE', ( #65476, #94682 ) ) ;
#103089=VERTEX_POINT ( 'NONE', #84657 ) ;
#103090=AXIS2_PLACEMENT_3D ( 'NONE', #4136, #64364, #12674 ) ;
#103091=CARTESIAN_POINT ( 'NONE',  ( -6.250000000000015987, 2.500000000000000000, 1.472243186433545459 ) ) ;
#103092=FACE_OUTER_BOUND ( 'NONE', #25507, .T. ) ;
#103094=LINE ( 'NONE', #63167, #60843 ) ;
#103095=CARTESIAN_POINT ( 'NONE',  ( -7.100000000000018296, 2.500000000000000000, 0.09999999999999761857 ) ) ;
#103096=CONICAL_SURFACE ( 'NONE', #4877, 0.1000000000000002554, 0.003490658503988666988 ) ;
#103097=ORIENTED_EDGE ( 'NONE', *, *, #69363, .T. ) ;
#103098=DIRECTION ( 'NONE',  ( -0.000000000000000000, -1.000000000000000000, -0.000000000000000000 ) ) ;
#103099=AXIS2_PLACEMENT_3D ( 'NONE', #22563, #122672, #62485 ) ;
#103100=AXIS2_PLACEMENT_3D ( 'NONE', #35445, #106106, #25596 ) ;
#103101=ORIENTED_EDGE ( 'NONE', *, *, #25448, .T. ) ;
#103102=CARTESIAN_POINT ( 'NONE',  ( 87.50000000000002842, 7.500000000000000000, -0.6928095518838441880 ) ) ;
#103103=EDGE_LOOP ( 'NONE', ( #14192, #93346 ) ) ;
#103104=DIRECTION ( 'NONE',  ( -4.274815082592931898E-19, -0.9999939076577903929, -0.003490651415223739937 ) ) ;
#103105=DIRECTION ( 'NONE',  ( 0.000000000000000000, 1.000000000000000000, 0.000000000000000000 ) ) ;
#103106=CARTESIAN_POINT ( 'NONE',  ( 8.749999999999957367, 2.500000000000000000, 2.265063509461097357 ) ) ;
#103107=LINE ( 'NONE', #53379, #73133 ) ;
#103108=CIRCLE ( 'NONE', #109369, 0.1000000000000000472 ) ;
#103109=ORIENTED_EDGE ( 'NONE', *, *, #85309, .T. ) ;
#103110=AXIS2_PLACEMENT_3D ( 'NONE', #109721, #29237, #39718 ) ;
#103111=CONICAL_SURFACE ( 'NONE', #52945, 0.1000000000000002554, 0.003490658503988666988 ) ;
#103112=DIRECTION ( 'NONE',  ( 0.000000000000000000, 1.000000000000000000, 0.000000000000000000 ) ) ;
#103113=CONICAL_SURFACE ( 'NONE', #9117, 0.1000000000000000472, 0.003490658503988666988 ) ;
#103114=EDGE_CURVE ( 'NONE', #82944, #23590, #82743, .T. ) ;
#103115=CARTESIAN_POINT ( 'NONE',  ( -1.250000000000036193, 2.500000000000000000, 1.472243186433545459 ) ) ;
#103116=EDGE_LOOP ( 'NONE', ( #119450, #64098 ) ) ;
#103117=ORIENTED_EDGE ( 'NONE', *, *, #81081, .F. ) ;
#103118=ORIENTED_EDGE ( 'NONE', *, *, #89463, .F. ) ;
#103119=DIRECTION ( 'NONE',  ( 0.000000000000000000, 0.000000000000000000, 1.000000000000000000 ) ) ;
#103120=CARTESIAN_POINT ( 'NONE',  ( -12.49999999999999467, 12.50000000000000000, 0.6928203230275535862 ) ) ;
#103122=CARTESIAN_POINT ( 'NONE',  ( 3.349999999999941913, 2.500000000000000000, 5.802370205355744659 ) ) ;
#103123=DIRECTION ( 'NONE',  ( 0.000000000000000000, -0.9999939076577903929, 0.003490651415223739937 ) ) ;
#103124=EDGE_CURVE ( 'NONE', #43713, #29164, #114749, .T. ) ;
#103125=CARTESIAN_POINT ( 'NONE',  ( 16.56576425165006583, 1.500000000000000888, -6.084390597445814564 ) ) ;
#103126=AXIS2_PLACEMENT_3D ( 'NONE', #51379, #127984, #28478 ) ;
#103127=CIRCLE ( 'NONE', #19493, 0.09999999999999982514 ) ;
#103128=CIRCLE ( 'NONE', #46693, 0.09999999999999999167 ) ;
#103129=LINE ( 'NONE', #12158, #88376 ) ;
#103131=ORIENTED_EDGE ( 'NONE', *, *, #94919, .F. ) ;
#103132=DIRECTION ( 'NONE',  ( 0.000000000000000000, 0.000000000000000000, 1.000000000000000000 ) ) ;
#103133=ORIENTED_EDGE ( 'NONE', *, *, #60515, .F. ) ;
#103134=DIRECTION ( 'NONE',  ( -0.000000000000000000, -1.000000000000000000, -0.000000000000000000 ) ) ;
#103135=DIRECTION ( 'NONE',  ( 0.000000000000000000, 1.000000000000000000, 0.000000000000000000 ) ) ;
#103136=DIRECTION ( 'NONE',  ( 0.000000000000000000, 1.000000000000000000, 0.000000000000000000 ) ) ;
#103137=DIRECTION ( 'NONE',  ( 0.000000000000000000, -0.000000000000000000, 1.000000000000000000 ) ) ;
#103138=VERTEX_POINT ( 'NONE', #110664 ) ;
#103139=DIRECTION ( 'NONE',  ( -0.000000000000000000, 1.000000000000000000, -0.000000000000000000 ) ) ;
#103140=CARTESIAN_POINT ( 'NONE',  ( 9.349999999999919709, 2.500000000000000000, -6.148780366869526226 ) ) ;
#103141=DIRECTION ( 'NONE',  ( 0.000000000000000000, 0.000000000000000000, 1.000000000000000000 ) ) ;
#103142=ORIENTED_EDGE ( 'NONE', *, *, #119280, .T. ) ;
#103143=AXIS2_PLACEMENT_3D ( 'NONE', #7784, #36631, #5840 ) ;
#103144=AXIS2_PLACEMENT_3D ( 'NONE', #7597, #47540, #28542 ) ;
#103145=EDGE_LOOP ( 'NONE', ( #15537, #27003, #1613, #61599 ) ) ;
#103146=DIRECTION ( 'NONE',  ( -4.274815082592931898E-19, -0.9999939076577903929, -0.003490651415223739937 ) ) ;
#103147=ADVANCED_FACE ( 'NONE', ( #81840 ), #52709, .T. ) ;
#103148=AXIS2_PLACEMENT_3D ( 'NONE', #127949, #37651, #58582 ) ;
#103149=AXIS2_PLACEMENT_3D ( 'NONE', #39396, #89752, #79308 ) ;
#103150=ORIENTED_EDGE ( 'NONE', *, *, #111799, .T. ) ;
#103151=AXIS2_PLACEMENT_3D ( 'NONE', #123629, #125564, #73898 ) ;
#103152=EDGE_LOOP ( 'NONE', ( #60566, #54898, #36692, #88671 ) ) ;
#103153=CARTESIAN_POINT ( 'NONE',  ( -3.550000000000028688, 2.500000000000000000, 6.841600689897072485 ) ) ;
#103154=AXIS2_PLACEMENT_3D ( 'NONE', #39566, #119369, #79474 ) ;
#103155=VERTEX_POINT ( 'NONE', #101505 ) ;
#103156=DIRECTION ( 'NONE',  ( 0.000000000000000000, 1.000000000000000000, 0.000000000000000000 ) ) ;
#103157=DIRECTION ( 'NONE',  ( -0.000000000000000000, 1.000000000000000000, -0.000000000000000000 ) ) ;
#103158=DIRECTION ( 'NONE',  ( 0.000000000000000000, 0.000000000000000000, 1.000000000000000000 ) ) ;
#103159=ADVANCED_FACE ( 'NONE', ( #90369 ), #710, .T. ) ;
#103160=CONICAL_SURFACE ( 'NONE', #71774, 0.1000000000000000472, 0.003490658503988666988 ) ;
#103161=ORIENTED_EDGE ( 'NONE', *, *, #51647, .T. ) ;
#103162=AXIS2_PLACEMENT_3D ( 'NONE', #38159, #59756, #29618 ) ;
#103163=DIRECTION ( 'NONE',  ( 0.000000000000000000, 0.000000000000000000, 1.000000000000000000 ) ) ;
#103164=CARTESIAN_POINT ( 'NONE',  ( -0.4000000000000392131, 12.50000000000000000, -5.022947341949754119 ) ) ;
#103165=CIRCLE ( 'NONE', #2821, 0.09999999999999982514 ) ;
#103166=VERTEX_POINT ( 'NONE', #30199 ) ;
#103167=AXIS2_PLACEMENT_3D ( 'NONE', #17101, #88447, #37442 ) ;
#103168=EDGE_CURVE ( 'NONE', #85752, #104158, #52797, .T. ) ;
#103170=CARTESIAN_POINT ( 'NONE',  ( -9.150000000000005684, 2.500000000000000000, 5.702370205355745014 ) ) ;
#103171=EDGE_CURVE ( 'NONE', #94866, #76, #71584, .T. ) ;
#103172=ORIENTED_EDGE ( 'NONE', *, *, #32022, .F. ) ;
#103173=EDGE_LOOP ( 'NONE', ( #46883, #115652 ) ) ;
#103174=EDGE_CURVE ( 'NONE', #120297, #91598, #60923, .T. ) ;
#103175=EDGE_LOOP ( 'NONE', ( #118373, #33301, #48044, #102725 ) ) ;
#103177=DIRECTION ( 'NONE',  ( 0.000000000000000000, 1.000000000000000000, 0.000000000000000000 ) ) ;
#103178=CARTESIAN_POINT ( 'NONE',  ( 11.84999999999990372, 2.500000000000000000, 1.818653347947321475 ) ) ;
#103179=DIRECTION ( 'NONE',  ( -0.000000000000000000, 1.000000000000000000, -0.000000000000000000 ) ) ;
#103180=EDGE_CURVE ( 'NONE', #44047, #32237, #92977, .T. ) ;
#103181=FACE_BOUND ( 'NONE', #18881, .T. ) ;
#103182=VERTEX_POINT ( 'NONE', #61592 ) ;
#103184=DIRECTION ( 'NONE',  ( 0.000000000000000000, 1.000000000000000000, 0.000000000000000000 ) ) ;
#103185=FACE_OUTER_BOUND ( 'NONE', #41281, .T. ) ;
#103186=DIRECTION ( 'NONE',  ( -0.000000000000000000, 1.000000000000000000, -0.000000000000000000 ) ) ;
#103187=DIRECTION ( 'NONE',  ( 0.000000000000000000, -0.9999939076577903929, 0.003490651415223739937 ) ) ;
#103188=CARTESIAN_POINT ( 'NONE',  ( -0.2000000000000408673, 2.500000000000000000, -3.883716857408426648 ) ) ;
#103189=CONICAL_SURFACE ( 'NONE', #63488, 0.1000000000000002554, 0.003490658503988666988 ) ;
#103190=VECTOR ( 'NONE', #59097, 1000.000000000000000 ) ;
#103191=DIRECTION ( 'NONE',  ( 0.000000000000000000, 0.000000000000000000, -1.000000000000000000 ) ) ;
#103193=ORIENTED_EDGE ( 'NONE', *, *, #8627, .F. ) ;
#103194=ORIENTED_EDGE ( 'NONE', *, *, #118879, .T. ) ;
#103195=ORIENTED_EDGE ( 'NONE', *, *, #68797, .T. ) ;
#103196=ORIENTED_EDGE ( 'NONE', *, *, #97036, .T. ) ;
#103197=CARTESIAN_POINT ( 'NONE',  ( 13.94999999999989271, 2.500000000000000000, -1.818653347947326138 ) ) ;
#103198=CARTESIAN_POINT ( 'NONE',  ( -0.8500000000000382805, 2.500000000000000000, -7.188010851410854052 ) ) ;
#103199=ORIENTED_EDGE ( 'NONE', *, *, #47244, .T. ) ;
#103200=FACE_BOUND ( 'NONE', #72009, .T. ) ;
#103201=CIRCLE ( 'NONE', #92747, 0.1000000000000002554 ) ;
#103202=CONICAL_SURFACE ( 'NONE', #27986, 0.1000000000000002554, 0.003490658503988666988 ) ;
#103203=CARTESIAN_POINT ( 'NONE',  ( 1.049999999999954525, 2.500000000000000000, 1.718653347947321386 ) ) ;
#103204=AXIS2_PLACEMENT_3D ( 'NONE', #3587, #15320, #65724 ) ;
#103205=AXIS2_PLACEMENT_3D ( 'NONE', #79639, #71110, #39748 ) ;
#103206=EDGE_CURVE ( 'NONE', #95333, #119700, #48605, .T. ) ;
#103207=EDGE_LOOP ( 'NONE', ( #32268, #124958, #94696, #94366 ) ) ;
#103208=DIRECTION ( 'NONE',  ( 0.000000000000000000, 0.000000000000000000, 1.000000000000000000 ) ) ;
#103209=CARTESIAN_POINT ( 'NONE',  ( 2.049999999999950084, 2.500000000000000000, -6.495190528383302464 ) ) ;
#103210=FACE_OUTER_BOUND ( 'NONE', #65372, .T. ) ;
#103211=CIRCLE ( 'NONE', #117866, 1.000000000000000888 ) ;
#103212=ORIENTED_EDGE ( 'NONE', *, *, #110128, .F. ) ;
#103214=EDGE_CURVE ( 'NONE', #42019, #17427, #62230, .T. ) ;
#103215=ORIENTED_EDGE ( 'NONE', *, *, #97095, .T. ) ;
#103216=CIRCLE ( 'NONE', #38492, 0.1000000000000000472 ) ;
#103217=AXIS2_PLACEMENT_3D ( 'NONE', #91206, #122604, #90555 ) ;
#103218=CIRCLE ( 'NONE', #94811, 0.06509327318403745899 ) ;
#103219=ORIENTED_EDGE ( 'NONE', *, *, #103821, .T. ) ;
#103220=ORIENTED_EDGE ( 'NONE', *, *, #11316, .T. ) ;
#103221=EDGE_CURVE ( 'NONE', #70284, #31342, #19339, .T. ) ;
#103222=DIRECTION ( 'NONE',  ( 0.000000000000000000, -0.000000000000000000, 1.000000000000000000 ) ) ;
#103223=CARTESIAN_POINT ( 'NONE',  ( -6.250000000000017764, 12.50000000000000000, 2.922977105672686982 ) ) ;
#103224=CARTESIAN_POINT ( 'NONE',  ( 3.349999999999945466, 2.500000000000000000, -7.288010851410854585 ) ) ;
#103225=AXIS2_PLACEMENT_3D ( 'NONE', #116084, #26427, #99028 ) ;
#103226=EDGE_CURVE ( 'NONE', #79060, #100871, #86231, .T. ) ;
#103227=ORIENTED_EDGE ( 'NONE', *, *, #42544, .T. ) ;
#103228=DIRECTION ( 'NONE',  ( 0.000000000000000000, 0.000000000000000000, -1.000000000000000000 ) ) ;
#103229=ADVANCED_FACE ( 'NONE', ( #50455 ), #29825, .T. ) ;
#103230=AXIS2_PLACEMENT_3D ( 'NONE', #49283, #77429, #117316 ) ;
#103231=CARTESIAN_POINT ( 'NONE',  ( 1.649999999999951505, 12.50000000000000000, -1.472243186433550122 ) ) ;
#103232=CARTESIAN_POINT ( 'NONE',  ( 11.24999999999991118, 2.500000000000000000, -2.857883832488653741 ) ) ;
#103233=EDGE_CURVE ( 'NONE', #890, #75136, #41946, .T. ) ;
#103235=ORIENTED_EDGE ( 'NONE', *, *, #53619, .T. ) ;
#103236=CARTESIAN_POINT ( 'NONE',  ( 5.799999999999931433, 12.50000000000000000, 4.330127018922196314 ) ) ;
#103237=ORIENTED_EDGE ( 'NONE', *, *, #40794, .T. ) ;
#103238=FACE_OUTER_BOUND ( 'NONE', #9982, .T. ) ;
#103239=EDGE_CURVE ( 'NONE', #14537, #11624, #102972, .T. ) ;
#103240=ADVANCED_FACE ( 'NONE', ( #41307 ), #72049, .T. ) ;
#103241=ORIENTED_EDGE ( 'NONE', *, *, #11430, .T. ) ;
#103242=ORIENTED_EDGE ( 'NONE', *, *, #23119, .F. ) ;
#103243=CARTESIAN_POINT ( 'NONE',  ( -4.150000000000024336, 2.500000000000000000, -2.165063509461101710 ) ) ;
#103244=DIRECTION ( 'NONE',  ( -0.000000000000000000, 1.000000000000000000, -0.000000000000000000 ) ) ;
#103245=CONICAL_SURFACE ( 'NONE', #835, 0.1000000000000002554, 0.003490658503988666988 ) ;
#103246=DIRECTION ( 'NONE',  ( 0.000000000000000000, -0.000000000000000000, 1.000000000000000000 ) ) ;
#103247=AXIS2_PLACEMENT_3D ( 'NONE', #107879, #67953, #47045 ) ;
#103248=FACE_OUTER_BOUND ( 'NONE', #90301, .T. ) ;
#103249=DIRECTION ( 'NONE',  ( 0.000000000000000000, 0.000000000000000000, -1.000000000000000000 ) ) ;
#103250=EDGE_LOOP ( 'NONE', ( #126770, #75527 ) ) ;
#103251=ORIENTED_EDGE ( 'NONE', *, *, #20919, .F. ) ;
#103253=CONICAL_SURFACE ( 'NONE', #117800, 0.1000000000000000472, 0.003490658503988666988 ) ;
#103254=CIRCLE ( 'NONE', #46822, 0.06509327318403741736 ) ;
#103255=DIRECTION ( 'NONE',  ( 0.000000000000000000, 0.000000000000000000, 1.000000000000000000 ) ) ;
#103256=AXIS2_PLACEMENT_3D ( 'NONE', #4224, #15327, #114197 ) ;
#103257=AXIS2_PLACEMENT_3D ( 'NONE', #41963, #92332, #89 ) ;
#103258=DIRECTION ( 'NONE',  ( 0.000000000000000000, 0.000000000000000000, -1.000000000000000000 ) ) ;
#103259=EDGE_LOOP ( 'NONE', ( #370, #28575, #93742, #44087 ) ) ;
#103260=VERTEX_POINT ( 'NONE', #111291 ) ;
#103261=CARTESIAN_POINT ( 'NONE',  ( 2.299999999999946976, 12.50000000000000000, 4.676537180435972552 ) ) ;
#103262=ORIENTED_EDGE ( 'NONE', *, *, #115585, .F. ) ;
#103263=DIRECTION ( 'NONE',  ( 0.000000000000000000, 1.000000000000000000, 0.000000000000000000 ) ) ;
#103264=CARTESIAN_POINT ( 'NONE',  ( 7.949999999999925571, 2.500000000000000000, 2.165063509461097713 ) ) ;
#103265=VECTOR ( 'NONE', #54218, 1000.000000000000000 ) ;
#103266=AXIS2_PLACEMENT_3D ( 'NONE', #85843, #16451, #6613 ) ;
#103267=VECTOR ( 'NONE', #58303, 1000.000000000000000 ) ;
#103268=DIRECTION ( 'NONE',  ( -0.000000000000000000, -1.000000000000000000, -0.000000000000000000 ) ) ;
#103269=VERTEX_POINT ( 'NONE', #22317 ) ;
#103270=FACE_OUTER_BOUND ( 'NONE', #9229, .T. ) ;
#103271=DIRECTION ( 'NONE',  ( -0.000000000000000000, 1.000000000000000000, -0.000000000000000000 ) ) ;
#103272=CARTESIAN_POINT ( 'NONE',  ( -3.550000000000031797, 2.500000000000000000, -6.148780366869526226 ) ) ;
#103273=FACE_OUTER_BOUND ( 'NONE', #70859, .T. ) ;
#103274=AXIS2_PLACEMENT_3D ( 'NONE', #15020, #42605, #72695 ) ;
#103275=CARTESIAN_POINT ( 'NONE',  ( -10.85000000000000142, 12.50000000000000000, -2.230156782645135394 ) ) ;
#103276=ORIENTED_EDGE ( 'NONE', *, *, #120900, .T. ) ;
#103277=CARTESIAN_POINT ( 'NONE',  ( 13.29999999999989946, 2.500000000000000000, -0.1000000000000023925 ) ) ;
#103278=ADVANCED_FACE ( 'NONE', ( #53048 ), #90433, .T. ) ;
#103279=CARTESIAN_POINT ( 'NONE',  ( -8.749999999999971578, 12.50000000000000000, 6.495190528383297135 ) ) ;
#103280=AXIS2_PLACEMENT_3D ( 'NONE', #18566, #38220, #27730 ) ;
#103281=ORIENTED_EDGE ( 'NONE', *, *, #16553, .F. ) ;
#103282=EDGE_LOOP ( 'NONE', ( #14661, #100272, #121604, #104580 ) ) ;
#103284=CARTESIAN_POINT ( 'NONE',  ( 8.149999999999923972, 12.50000000000000000, 2.576566944158910744 ) ) ;
#103285=CARTESIAN_POINT ( 'NONE',  ( 9.599999999999914380, 2.500000000000000000, 4.430127018922196847 ) ) ;
#103286=CIRCLE ( 'NONE', #69825, 0.09999999999999982514 ) ;
#103287=FACE_OUTER_BOUND ( 'NONE', #24822, .T. ) ;
#103288=DIRECTION ( 'NONE',  ( 0.000000000000000000, 0.000000000000000000, 1.000000000000000000 ) ) ;
#103289=ADVANCED_FACE ( 'NONE', ( #70113 ), #13070, .T. ) ;
#103290=LINE ( 'NONE', #53545, #32523 ) ;
#103291=DIRECTION ( 'NONE',  ( 0.000000000000000000, 0.000000000000000000, -1.000000000000000000 ) ) ;
#103293=DIRECTION ( 'NONE',  ( 0.000000000000000000, 0.000000000000000000, 1.000000000000000000 ) ) ;
#103294=DIRECTION ( 'NONE',  ( 0.000000000000000000, 1.000000000000000000, 0.000000000000000000 ) ) ;
#103296=CONICAL_SURFACE ( 'NONE', #107493, 0.1000000000000002554, 0.003490658503988666988 ) ;
#103297=EDGE_LOOP ( 'NONE', ( #88089, #105396, #69123, #21672 ) ) ;
#103298=CIRCLE ( 'NONE', #48922, 0.06509327318403745899 ) ;
#103299=EDGE_LOOP ( 'NONE', ( #84187, #2941 ) ) ;
#103300=EDGE_LOOP ( 'NONE', ( #105748, #39484, #3990, #96642 ) ) ;
#103301=ORIENTED_EDGE ( 'NONE', *, *, #68155, .F. ) ;
#103302=CONICAL_SURFACE ( 'NONE', #40331, 0.1000000000000000056, 0.003490658503988666988 ) ;
#103303=CARTESIAN_POINT ( 'NONE',  ( -11.04999999999999893, 12.50000000000000000, 6.148780366869520009 ) ) ;
#103304=DIRECTION ( 'NONE',  ( 0.000000000000000000, 1.000000000000000000, 0.000000000000000000 ) ) ;
#103305=ORIENTED_EDGE ( 'NONE', *, *, #61396, .F. ) ;
#103306=DIRECTION ( 'NONE',  ( -0.000000000000000000, 1.000000000000000000, -0.000000000000000000 ) ) ;
#103307=AXIS2_PLACEMENT_3D ( 'NONE', #61801, #19936, #59882 ) ;
#103308=DIRECTION ( 'NONE',  ( 0.000000000000000000, 1.000000000000000000, 0.000000000000000000 ) ) ;
#103309=CARTESIAN_POINT ( 'NONE',  ( -2.900000000000029221, 2.500000000000000000, -5.122947341949753763 ) ) ;
#103311=DIRECTION ( 'NONE',  ( 0.000000000000000000, 0.000000000000000000, 1.000000000000000000 ) ) ;
#103312=CARTESIAN_POINT ( 'NONE',  ( 4.349999999999940137, 2.500000000000000000, -2.511473670974877948 ) ) ;
#103313=VERTEX_POINT ( 'NONE', #10523 ) ;
#103314=CIRCLE ( 'NONE', #9307, 0.09999999999999982514 ) ;
#103315=CIRCLE ( 'NONE', #90785, 0.06509327318403745899 ) ;
#103316=EDGE_LOOP ( 'NONE', ( #115768, #123703, #43235, #69719 ) ) ;
#103317=ORIENTED_EDGE ( 'NONE', *, *, #16355, .F. ) ;
#103318=VERTEX_POINT ( 'NONE', #123688 ) ;
#103319=CARTESIAN_POINT ( 'NONE',  ( 9.999999999999912959, 2.500000000000000000, -4.922947341949753586 ) ) ;
#103320=AXIS2_PLACEMENT_3D ( 'NONE', #72794, #51237, #121883 ) ;
#103321=DIRECTION ( 'NONE',  ( 0.000000000000000000, -0.000000000000000000, 1.000000000000000000 ) ) ;
#103322=DIRECTION ( 'NONE',  ( 0.000000000000000000, 0.000000000000000000, 1.000000000000000000 ) ) ;
#103323=CIRCLE ( 'NONE', #23909, 0.06509327318403745899 ) ;
#103325=EDGE_CURVE ( 'NONE', #54263, #89280, #88284, .T. ) ;
#103326=ORIENTED_EDGE ( 'NONE', *, *, #67717, .T. ) ;
#103327=CARTESIAN_POINT ( 'NONE',  ( -11.05000000000000071, 12.50000000000000000, -2.446380397790836270 ) ) ;
#103328=EDGE_LOOP ( 'NONE', ( #15239, #18916 ) ) ;
#103330=DIRECTION ( 'NONE',  ( 0.000000000000000000, 0.000000000000000000, 1.000000000000000000 ) ) ;
#103331=EDGE_CURVE ( 'NONE', #7558, #73190, #63263, .T. ) ;
#103332=DIRECTION ( 'NONE',  ( -4.274815082592931898E-19, -0.9999939076577903929, -0.003490651415223739937 ) ) ;
#103333=DIRECTION ( 'NONE',  ( 0.000000000000000000, 1.000000000000000000, 0.000000000000000000 ) ) ;
#103334=EDGE_CURVE ( 'NONE', #93212, #11168, #17265, .T. ) ;
#103335=ORIENTED_EDGE ( 'NONE', *, *, #59304, .F. ) ;
#103336=AXIS2_PLACEMENT_3D ( 'NONE', #27584, #106794, #17100 ) ;
#103337=EDGE_LOOP ( 'NONE', ( #67491, #65895, #59711, #77232 ) ) ;
#103338=ADVANCED_FACE ( 'NONE', ( #54330 ), #83783, .T. ) ;
#103339=CIRCLE ( 'NONE', #86592, 0.06509327318403741736 ) ;
#103340=EDGE_CURVE ( 'NONE', #6261, #54499, #113905, .T. ) ;
#103341=ORIENTED_EDGE ( 'NONE', *, *, #31895, .F. ) ;
#103342=LINE ( 'NONE', #102049, #7179 ) ;
#103343=CARTESIAN_POINT ( 'NONE',  ( 7.899999999999923084, 12.50000000000000000, -0.6928203230275542523 ) ) ;
#103344=CIRCLE ( 'NONE', #122124, 0.06509327318403745899 ) ;
#103345=AXIS2_PLACEMENT_3D ( 'NONE', #494, #12251, #40459 ) ;
#103346=CARTESIAN_POINT ( 'NONE',  ( -8.350000000000012079, 2.500000000000000000, -1.472243186433550122 ) ) ;
#103347=ADVANCED_FACE ( 'NONE', ( #54965 ), #107167, .T. ) ;
#103348=FACE_BOUND ( 'NONE', #65773, .T. ) ;
#103349=DIRECTION ( 'NONE',  ( 0.000000000000000000, 1.000000000000000000, 0.000000000000000000 ) ) ;
#103350=DIRECTION ( 'NONE',  ( 0.000000000000000000, 0.000000000000000000, 1.000000000000000000 ) ) ;
#103351=DIRECTION ( 'NONE',  ( 0.000000000000000000, 0.000000000000000000, 1.000000000000000000 ) ) ;
#103352=CIRCLE ( 'NONE', #46917, 0.1000000000000002554 ) ;
#103353=CIRCLE ( 'NONE', #105494, 0.06509327318403745899 ) ;
#103354=VECTOR ( 'NONE', #36316, 1000.000000000000000 ) ;
#103355=CARTESIAN_POINT ( 'NONE',  ( 2.500000000000002220, 2.500000000000000000, 9.000000000000003553 ) ) ;
#103356=FACE_OUTER_BOUND ( 'NONE', #118888, .T. ) ;
#103357=DIRECTION ( 'NONE',  ( 0.000000000000000000, -0.000000000000000000, 1.000000000000000000 ) ) ;
#103358=VERTEX_POINT ( 'NONE', #45808 ) ;
#103359=VECTOR ( 'NONE', #37793, 1000.000000000000000 ) ;
#103360=AXIS2_PLACEMENT_3D ( 'NONE', #77193, #109213, #58842 ) ;
#103361=VECTOR ( 'NONE', #42535, 1000.000000000000000 ) ;
#103362=LINE ( 'NONE', #5138, #5680 ) ;
#103363=ORIENTED_EDGE ( 'NONE', *, *, #108983, .F. ) ;
#103364=VERTEX_POINT ( 'NONE', #84434 ) ;
#103365=DIRECTION ( 'NONE',  ( 0.000000000000000000, 1.000000000000000000, 0.000000000000000000 ) ) ;
#103366=FACE_BOUND ( 'NONE', #104999, .T. ) ;
#103367=LINE ( 'NONE', #113170, #84961 ) ;
#103368=EDGE_LOOP ( 'NONE', ( #110815, #50946 ) ) ;
#103369=CARTESIAN_POINT ( 'NONE',  ( 23.85240649353447751, 2.660544618071316147, 4.258220037268930724 ) ) ;
#103370=FACE_OUTER_BOUND ( 'NONE', #78666, .T. ) ;
#103371=ORIENTED_EDGE ( 'NONE', *, *, #61010, .F. ) ;
#103372=DIRECTION ( 'NONE',  ( 0.000000000000000000, 1.000000000000000000, 0.000000000000000000 ) ) ;
#103373=CARTESIAN_POINT ( 'NONE',  ( -3.749999999999994671, 2.500000000000000000, -6.595190528383302109 ) ) ;
#103374=EDGE_CURVE ( 'NONE', #81926, #118944, #21402, .T. ) ;
#103375=ORIENTED_EDGE ( 'NONE', *, *, #45549, .F. ) ;
#103376=EDGE_CURVE ( 'NONE', #43898, #118209, #75776, .T. ) ;
#103377=CARTESIAN_POINT ( 'NONE',  ( -6.050000000000017586, 12.50000000000000000, 1.883746621131358934 ) ) ;
#103378=CARTESIAN_POINT ( 'NONE',  ( -6.050000000000018474, 12.50000000000000000, 6.841600689897072485 ) ) ;
#103379=ADVANCED_FACE ( 'NONE', ( #125001 ), #105018, .T. ) ;
#103380=AXIS2_PLACEMENT_3D ( 'NONE', #6273, #46218, #86119 ) ;
#103381=ORIENTED_EDGE ( 'NONE', *, *, #43425, .T. ) ;
#103382=DIRECTION ( 'NONE',  ( -0.000000000000000000, -1.000000000000000000, -0.000000000000000000 ) ) ;
#103383=CARTESIAN_POINT ( 'NONE',  ( 0.5999999999999612310, 2.500000000000000000, -0.3464101615137760715 ) ) ;
#103384=PLANE ( 'NONE',  #47217 ) ;
#103385=ADVANCED_FACE ( 'NONE', ( #34716 ), #117611, .T. ) ;
#103387=EDGE_LOOP ( 'NONE', ( #63400, #98559, #27090, #113664 ) ) ;
#103388=ORIENTED_EDGE ( 'NONE', *, *, #103781, .F. ) ;
#103389=ADVANCED_FACE ( 'NONE', ( #53687 ), #65305, .T. ) ;
#103391=EDGE_LOOP ( 'NONE', ( #79103, #60803, #11945, #31967 ) ) ;
#103392=CARTESIAN_POINT ( 'NONE',  ( 4.399999999999940847, 12.50000000000000000, -4.611443907251939756 ) ) ;
#103393=CARTESIAN_POINT ( 'NONE',  ( 5.649999999999934630, 12.50000000000000000, 6.083687093685483660 ) ) ;
#103394=ADVANCED_FACE ( 'NONE', ( #93608 ), #8871, .T. ) ;
#103395=AXIS2_PLACEMENT_3D ( 'NONE', #52601, #42822, #74185 ) ;
#103396=ADVANCED_FACE ( 'NONE', ( #64143 ), #105364, .F. ) ;
#103397=ORIENTED_EDGE ( 'NONE', *, *, #37475, .F. ) ;
#103398=CARTESIAN_POINT ( 'NONE',  ( 9.599999999999914380, 2.500000000000000000, -4.330127018922201643 ) ) ;
#103399=CARTESIAN_POINT ( 'NONE',  ( -9.600000000000008527, 12.50000000000000000, 4.265033745738159077 ) ) ;
#103400=CARTESIAN_POINT ( 'NONE',  ( -1.650000000000035216, 2.500000000000000000, -5.902370205355750521 ) ) ;
#103401=DIRECTION ( 'NONE',  ( 0.000000000000000000, 1.000000000000000000, 0.000000000000000000 ) ) ;
#103402=CARTESIAN_POINT ( 'NONE',  ( -10.00000000000000533, 12.50000000000000000, -4.957854068765712441 ) ) ;
#103403=EDGE_CURVE ( 'NONE', #3528, #11005, #98763, .T. ) ;
#103404=VERTEX_POINT ( 'NONE', #96174 ) ;
#103405=ORIENTED_EDGE ( 'NONE', *, *, #11627, .F. ) ;
#103406=DIRECTION ( 'NONE',  ( 0.000000000000000000, 0.000000000000000000, 1.000000000000000000 ) ) ;
#103407=VECTOR ( 'NONE', #97230, 1000.000000000000000 ) ;
#103408=CIRCLE ( 'NONE', #63704, 0.06509327318403745899 ) ;
#103410=EDGE_LOOP ( 'NONE', ( #104729, #37915 ) ) ;
#103411=ORIENTED_EDGE ( 'NONE', *, *, #47010, .T. ) ;
#103412=ORIENTED_EDGE ( 'NONE', *, *, #51487, .F. ) ;
#103414=CARTESIAN_POINT ( 'NONE',  ( -2.050000000000032685, 12.50000000000000000, -2.230156782645139391 ) ) ;
#103415=CIRCLE ( 'NONE', #105465, 0.06509327318403741736 ) ;
#103416=LINE ( 'NONE', #43222, #119602 ) ;
#103417=DIRECTION ( 'NONE',  ( 0.000000000000000000, 0.000000000000000000, 1.000000000000000000 ) ) ;
#103419=CARTESIAN_POINT ( 'NONE',  ( 2.500000000000002220, -1.500000000000000000, 10.00000000000000178 ) ) ;
#103420=CARTESIAN_POINT ( 'NONE',  ( 1.049999999999954525, 2.500000000000000000, 1.818653347947321475 ) ) ;
#103421=DIRECTION ( 'NONE',  ( 0.000000000000000000, -0.9999939076577903929, 0.003490651415223739937 ) ) ;
#103422=DIRECTION ( 'NONE',  ( 0.000000000000000000, 0.000000000000000000, -1.000000000000000000 ) ) ;
#103423=CARTESIAN_POINT ( 'NONE',  ( 10.64999999999990976, 2.500000000000000000, -6.148780366869526226 ) ) ;
#103424=FACE_OUTER_BOUND ( 'NONE', #65894, .T. ) ;
#103425=VERTEX_POINT ( 'NONE', #14385 ) ;
#103426=CIRCLE ( 'NONE', #107626, 0.06509327318403745899 ) ;
#103427=CIRCLE ( 'NONE', #46998, 0.06509327318403745899 ) ;
#103428=FACE_OUTER_BOUND ( 'NONE', #123495, .T. ) ;
#103429=AXIS2_PLACEMENT_3D ( 'NONE', #120023, #129224, #38915 ) ;
#103430=VECTOR ( 'NONE', #6926, 1000.000000000000000 ) ;
#103431=EDGE_LOOP ( 'NONE', ( #15324, #108687, #37946, #43367 ) ) ;
#103432=ORIENTED_EDGE ( 'NONE', *, *, #94169, .F. ) ;
#103434=DIRECTION ( 'NONE',  ( 0.000000000000000000, 0.000000000000000000, 1.000000000000000000 ) ) ;
#103435=DIRECTION ( 'NONE',  ( -0.000000000000000000, -1.000000000000000000, -0.000000000000000000 ) ) ;
#103436=VECTOR ( 'NONE', #48203, 1000.000000000000000 ) ;
#103437=DIRECTION ( 'NONE',  ( 0.000000000000000000, 0.000000000000000000, 1.000000000000000000 ) ) ;
#103438=EDGE_CURVE ( 'NONE', #53090, #93141, #43885, .T. ) ;
#103439=AXIS2_PLACEMENT_3D ( 'NONE', #113192, #34006, #23528 ) ;
#103440=CIRCLE ( 'NONE', #38714, 0.1000000000000000472 ) ;
#103441=DIRECTION ( 'NONE',  ( 0.000000000000000000, -0.9999939076577903929, 0.003490651415223739937 ) ) ;
#103443=DIRECTION ( 'NONE',  ( 0.000000000000000000, 0.000000000000000000, -1.000000000000000000 ) ) ;
#103444=VERTEX_POINT ( 'NONE', #106647 ) ;
#103445=DIRECTION ( 'NONE',  ( 0.000000000000000000, 0.000000000000000000, 1.000000000000000000 ) ) ;
#103446=AXIS2_PLACEMENT_3D ( 'NONE', #75760, #98610, #58079 ) ;
#103448=AXIS2_PLACEMENT_3D ( 'NONE', #15521, #54804, #94735 ) ;
#103449=ORIENTED_EDGE ( 'NONE', *, *, #66003, .T. ) ;
#103450=AXIS2_PLACEMENT_3D ( 'NONE', #92246, #62805, #102704 ) ;
#103451=ORIENTED_EDGE ( 'NONE', *, *, #104526, .T. ) ;
#103452=ORIENTED_EDGE ( 'NONE', *, *, #87822, .T. ) ;
#103453=CIRCLE ( 'NONE', #49085, 0.09999999999999982514 ) ;
#103454=VERTEX_POINT ( 'NONE', #39237 ) ;
#103455=DIRECTION ( 'NONE',  ( 0.000000000000000000, 1.000000000000000000, 0.000000000000000000 ) ) ;
#103456=CARTESIAN_POINT ( 'NONE',  ( 6.699999999999930012, 2.500000000000000000, 4.430127018922196847 ) ) ;
#103457=CARTESIAN_POINT ( 'NONE',  ( 14.34999999999989662, 2.500000000000000000, 2.611473670974873151 ) ) ;
#103458=CARTESIAN_POINT ( 'NONE',  ( 7.099999999999928590, 2.500000000000000000, -4.430127018922202176 ) ) ;
#103459=CARTESIAN_POINT ( 'NONE',  ( -7.700000000000012612, 2.500000000000000000, 4.676537180435972552 ) ) ;
#103460=ORIENTED_EDGE ( 'NONE', *, *, #51546, .T. ) ;
#103461=CARTESIAN_POINT ( 'NONE',  ( 32.27737262862851964, -1.406459147574385504, 4.686451386305379607 ) ) ;
#103462=DIRECTION ( 'NONE',  ( -0.000000000000000000, 1.000000000000000000, -0.000000000000000000 ) ) ;
#103463=DIRECTION ( 'NONE',  ( 0.000000000000000000, -0.9999939076577903929, 0.003490651415223739937 ) ) ;
#103464=CIRCLE ( 'NONE', #76270, 0.06509327318403745899 ) ;
#103465=CARTESIAN_POINT ( 'NONE',  ( -9.150000000000009237, 2.500000000000000000, -6.495190528383297135 ) ) ;
#103466=ORIENTED_EDGE ( 'NONE', *, *, #43501, .T. ) ;
#103467=VERTEX_POINT ( 'NONE', #27429 ) ;
#103468=ORIENTED_EDGE ( 'NONE', *, *, #49808, .F. ) ;
#103469=CARTESIAN_POINT ( 'NONE',  ( 0.3999999999999619971, 2.500000000000000000, -0.1000000000000001166 ) ) ;
#103470=CONICAL_SURFACE ( 'NONE', #95155, 0.09999999999999982514, 0.003490658503988666988 ) ;
#103471=DIRECTION ( 'NONE',  ( -0.000000000000000000, 1.000000000000000000, -0.000000000000000000 ) ) ;
#103472=CARTESIAN_POINT ( 'NONE',  ( -14.39999999999998614, 2.500000000000000000, -0.4464101615137760493 ) ) ;
#103473=VECTOR ( 'NONE', #111049, 1000.000000000000000 ) ;
#103474=EDGE_CURVE ( 'NONE', #49409, #70661, #2613, .T. ) ;
#103475=ORIENTED_EDGE ( 'NONE', *, *, #102803, .F. ) ;
#103476=LINE ( 'NONE', #104121, #51580 ) ;
#103477=CARTESIAN_POINT ( 'NONE',  ( 10.19999999999991580, 2.500000000000000000, -0.3464101615137783474 ) ) ;
#103478=EDGE_CURVE ( 'NONE', #14553, #52245, #107290, .T. ) ;
#103479=CARTESIAN_POINT ( 'NONE',  ( -12.49999999999999289, 12.50000000000000000, -0.6277270498435125745 ) ) ;
#103480=LINE ( 'NONE', #115196, #79135 ) ;
#103481=EDGE_CURVE ( 'NONE', #460, #4381, #126945, .T. ) ;
#103482=CARTESIAN_POINT ( 'NONE',  ( -10.80000000000000071, 2.500000000000000000, 4.330127018922196314 ) ) ;
#103483=AXIS2_PLACEMENT_3D ( 'NONE', #25428, #113842, #24164 ) ;
#103484=ORIENTED_EDGE ( 'NONE', *, *, #88816, .T. ) ;
#103485=EDGE_CURVE ( 'NONE', #21052, #115754, #69515, .T. ) ;
#103486=EDGE_CURVE ( 'NONE', #21966, #81870, #121842, .T. ) ;
#103487=ORIENTED_EDGE ( 'NONE', *, *, #29630, .T. ) ;
#103488=EDGE_CURVE ( 'NONE', #3295, #13562, #29918, .T. ) ;
#103490=EDGE_CURVE ( 'NONE', #88669, #42865, #26187, .T. ) ;
#103491=EDGE_CURVE ( 'NONE', #92653, #106656, #58843, .T. ) ;
#103492=DIRECTION ( 'NONE',  ( -0.000000000000000000, 1.000000000000000000, -0.000000000000000000 ) ) ;
#103493=DIRECTION ( 'NONE',  ( 0.000000000000000000, 1.000000000000000000, 0.000000000000000000 ) ) ;
#103494=DIRECTION ( 'NONE',  ( 0.000000000000000000, 1.000000000000000000, 0.000000000000000000 ) ) ;
#103495=CARTESIAN_POINT ( 'NONE',  ( 0.6499999999999543920, 12.50000000000000000, 6.148780366869520897 ) ) ;
#103496=ORIENTED_EDGE ( 'NONE', *, *, #51888, .T. ) ;
#103497=AXIS2_PLACEMENT_3D ( 'NONE', #108960, #960, #60556 ) ;
#103498=CIRCLE ( 'NONE', #15643, 0.06509327318403745899 ) ;
#103499=VERTEX_POINT ( 'NONE', #48378 ) ;
#103500=CARTESIAN_POINT ( 'NONE',  ( 8.299999999999922551, 12.50000000000000000, 4.395220292106234439 ) ) ;
#103501=LINE ( 'NONE', #13808, #44705 ) ;
#103502=EDGE_CURVE ( 'NONE', #106434, #109438, #84286, .T. ) ;
#103503=CARTESIAN_POINT ( 'NONE',  ( 17.99892161670943480, -2.500000000000000444, -4.934975022999348759 ) ) ;
#103504=DIRECTION ( 'NONE',  ( 0.000000000000000000, 1.000000000000000000, 0.000000000000000000 ) ) ;
#103505=ORIENTED_EDGE ( 'NONE', *, *, #77746, .F. ) ;
#103506=DIRECTION ( 'NONE',  ( 0.000000000000000000, -0.000000000000000000, 1.000000000000000000 ) ) ;
#103507=EDGE_CURVE ( 'NONE', #80752, #76477, #61313, .T. ) ;
#103508=DIRECTION ( 'NONE',  ( 0.000000000000000000, 0.000000000000000000, -1.000000000000000000 ) ) ;
#103509=EDGE_LOOP ( 'NONE', ( #125413, #85453, #87036, #44618 ) ) ;
#103510=DIRECTION ( 'NONE',  ( 0.000000000000000000, 0.000000000000000000, -1.000000000000000000 ) ) ;
#103511=AXIS2_PLACEMENT_3D ( 'NONE', #91024, #22933, #102759 ) ;
#103513=DIRECTION ( 'NONE',  ( 0.000000000000000000, 0.000000000000000000, 1.000000000000000000 ) ) ;
#103514=AXIS2_PLACEMENT_3D ( 'NONE', #62727, #63358, #124210 ) ;
#103516=CARTESIAN_POINT ( 'NONE',  ( -4.150000000000024336, 12.50000000000000000, -2.857883832488653741 ) ) ;
#103517=CARTESIAN_POINT ( 'NONE',  ( -0.8500000000000386136, 12.50000000000000000, 5.802370205355744659 ) ) ;
#103518=CONICAL_SURFACE ( 'NONE', #118179, 0.09999999999999982514, 0.003490658503988666988 ) ;
#103519=AXIS2_PLACEMENT_3D ( 'NONE', #70081, #40643, #107419 ) ;
#103520=ORIENTED_EDGE ( 'NONE', *, *, #69353, .F. ) ;
#103521=ORIENTED_EDGE ( 'NONE', *, *, #8944, .F. ) ;
#103523=FACE_OUTER_BOUND ( 'NONE', #109190, .T. ) ;
#103526=AXIS2_PLACEMENT_3D ( 'NONE', #43400, #32943, #75404 ) ;
#103527=AXIS2_PLACEMENT_3D ( 'NONE', #69243, #97423, #7752 ) ;
#103528=CIRCLE ( 'NONE', #97258, 0.06509327318403745899 ) ;
#103529=LINE ( 'NONE', #51219, #68136 ) ;
#103530=CARTESIAN_POINT ( 'NONE',  ( -13.09999999999999254, 2.500000000000000000, -0.4464101615137741064 ) ) ;
#103531=CIRCLE ( 'NONE', #86794, 0.09999999999999982514 ) ;
#103532=CARTESIAN_POINT ( 'NONE',  ( -7.900000000000011013, 12.50000000000000000, 5.022947341949748790 ) ) ;
#103533=ADVANCED_FACE ( 'NONE', ( #37907 ), #126297, .T. ) ;
#103534=CARTESIAN_POINT ( 'NONE',  ( -13.74999999999998757, 12.50000000000000000, 1.472243186433549456 ) ) ;
#103535=EDGE_CURVE ( 'NONE', #15950, #22180, #87005, .T. ) ;
#103536=AXIS2_PLACEMENT_3D ( 'NONE', #115497, #52729, #25193 ) ;
#103537=CIRCLE ( 'NONE', #109797, 0.06509327318403745899 ) ;
#103538=VERTEX_POINT ( 'NONE', #9091 ) ;
#103539=EDGE_CURVE ( 'NONE', #40733, #99388, #42451, .T. ) ;
#103540=ORIENTED_EDGE ( 'NONE', *, *, #27522, .F. ) ;
#103541=DIRECTION ( 'NONE',  ( 0.000000000000000000, 0.000000000000000000, 1.000000000000000000 ) ) ;
#103542=ORIENTED_EDGE ( 'NONE', *, *, #22733, .F. ) ;
#103544=DIRECTION ( 'NONE',  ( 0.000000000000000000, 1.000000000000000000, 0.000000000000000000 ) ) ;
#103545=AXIS2_PLACEMENT_3D ( 'NONE', #127131, #57072, #19751 ) ;
#103546=DIRECTION ( 'NONE',  ( 0.000000000000000000, 0.000000000000000000, 1.000000000000000000 ) ) ;
#103547=VERTEX_POINT ( 'NONE', #29396 ) ;
#103548=VERTEX_POINT ( 'NONE', #96819 ) ;
#103549=CARTESIAN_POINT ( 'NONE',  ( 6.249999999999930722, 2.500000000000000000, -1.572243186433550211 ) ) ;
#103550=ORIENTED_EDGE ( 'NONE', *, *, #44534, .T. ) ;
#103551=EDGE_CURVE ( 'NONE', #22696, #58191, #21508, .T. ) ;
#103552=DIRECTION ( 'NONE',  ( -0.000000000000000000, -1.000000000000000000, -0.000000000000000000 ) ) ;
#103553=CARTESIAN_POINT ( 'NONE',  ( -10.85000000000000142, 2.500000000000000000, 2.165063509461097713 ) ) ;
#103554=EDGE_CURVE ( 'NONE', #121714, #82618, #46636, .T. ) ;
#103555=FACE_OUTER_BOUND ( 'NONE', #101511, .T. ) ;
#103556=DIRECTION ( 'NONE',  ( 0.000000000000000000, 0.000000000000000000, -1.000000000000000000 ) ) ;
#103557=DIRECTION ( 'NONE',  ( 0.000000000000000000, 1.000000000000000000, 0.000000000000000000 ) ) ;
#103558=EDGE_CURVE ( 'NONE', #20569, #31101, #92611, .T. ) ;
#103559=DIRECTION ( 'NONE',  ( 0.000000000000000000, 0.000000000000000000, -1.000000000000000000 ) ) ;
#103560=CARTESIAN_POINT ( 'NONE',  ( -12.89999999999999325, 12.50000000000000000, -3.702399969078684627 ) ) ;
#103561=LINE ( 'NONE', #64261, #5576 ) ;
#103562=DIRECTION ( 'NONE',  ( -0.000000000000000000, -1.000000000000000000, -0.000000000000000000 ) ) ;
#103563=DIRECTION ( 'NONE',  ( 0.000000000000000000, 0.000000000000000000, -1.000000000000000000 ) ) ;
#103564=AXIS2_PLACEMENT_3D ( 'NONE', #5319, #15783, #45266 ) ;
#103565=CARTESIAN_POINT ( 'NONE',  ( -9.400000000000009237, 2.500000000000000000, -4.576537180435973795 ) ) ;
#103566=EDGE_CURVE ( 'NONE', #40625, #25430, #77196, .T. ) ;
#103567=VERTEX_POINT ( 'NONE', #97475 ) ;
#103568=ORIENTED_EDGE ( 'NONE', *, *, #123934, .F. ) ;
#103569=VERTEX_POINT ( 'NONE', #28940 ) ;
#103570=DIRECTION ( 'NONE',  ( -0.000000000000000000, 1.000000000000000000, -0.000000000000000000 ) ) ;
#103571=ORIENTED_EDGE ( 'NONE', *, *, #23719, .T. ) ;
#103572=DIRECTION ( 'NONE',  ( 0.000000000000000000, 1.000000000000000000, 0.000000000000000000 ) ) ;
#103573=VERTEX_POINT ( 'NONE', #107490 ) ;
#103574=EDGE_LOOP ( 'NONE', ( #34366, #77587 ) ) ;
#103575=ORIENTED_EDGE ( 'NONE', *, *, #43683, .T. ) ;
#103576=DIRECTION ( 'NONE',  ( -0.000000000000000000, -1.000000000000000000, -0.000000000000000000 ) ) ;
#103577=AXIS2_PLACEMENT_3D ( 'NONE', #116097, #126572, #95814 ) ;
#103578=VECTOR ( 'NONE', #51524, 1000.000000000000000 ) ;
#103579=DIRECTION ( 'NONE',  ( 0.000000000000000000, 1.000000000000000000, 0.000000000000000000 ) ) ;
#103582=DIRECTION ( 'NONE',  ( -0.000000000000000000, -1.000000000000000000, -0.000000000000000000 ) ) ;
#103583=CARTESIAN_POINT ( 'NONE',  ( 4.599999999999940137, 2.500000000000000000, -5.022947341949754119 ) ) ;
#103584=EDGE_CURVE ( 'NONE', #96634, #127530, #38242, .T. ) ;
#103585=ORIENTED_EDGE ( 'NONE', *, *, #3499, .F. ) ;
#103586=LINE ( 'NONE', #94386, #122945 ) ;
#103587=VERTEX_POINT ( 'NONE', #69483 ) ;
#103588=CIRCLE ( 'NONE', #72198, 0.06509327318403745899 ) ;
#103589=ORIENTED_EDGE ( 'NONE', *, *, #28267, .T. ) ;
#103590=ORIENTED_EDGE ( 'NONE', *, *, #34949, .T. ) ;
#103591=VECTOR ( 'NONE', #120918, 1000.000000000000000 ) ;
#103592=DIRECTION ( 'NONE',  ( -0.000000000000000000, 1.000000000000000000, -0.000000000000000000 ) ) ;
#103593=EDGE_LOOP ( 'NONE', ( #30504, #24796 ) ) ;
#103594=ORIENTED_EDGE ( 'NONE', *, *, #33628, .F. ) ;
#103595=ORIENTED_EDGE ( 'NONE', *, *, #60657, .F. ) ;
#103596=DIRECTION ( 'NONE',  ( -4.274815082592931898E-19, -0.9999939076577903929, -0.003490651415223739937 ) ) ;
#103597=DIRECTION ( 'NONE',  ( -0.000000000000000000, 1.000000000000000000, -0.000000000000000000 ) ) ;
#103598=VECTOR ( 'NONE', #104164, 1000.000000000000000 ) ;
#103599=CARTESIAN_POINT ( 'NONE',  ( -5.600000000000020073, 12.50000000000000000, 3.983716857408420964 ) ) ;
#103600=AXIS2_PLACEMENT_3D ( 'NONE', #103709, #54578, #95810 ) ;
#103601=EDGE_CURVE ( 'NONE', #39180, #116552, #88373, .T. ) ;
#103602=DIRECTION ( 'NONE',  ( 0.000000000000000000, 0.000000000000000000, 1.000000000000000000 ) ) ;
#103603=CARTESIAN_POINT ( 'NONE',  ( -3.950000000000024603, 2.500000000000000000, 1.818653347947321475 ) ) ;
#103604=CARTESIAN_POINT ( 'NONE',  ( -5.450000000000019718, 2.500000000000000000, 2.165063509461097713 ) ) ;
#103605=DIRECTION ( 'NONE',  ( 0.000000000000000000, 0.000000000000000000, 1.000000000000000000 ) ) ;
#103606=ORIENTED_EDGE ( 'NONE', *, *, #41947, .F. ) ;
#103607=CARTESIAN_POINT ( 'NONE',  ( -1.250000000000001110, 12.50000000000000000, -2.165063509461101710 ) ) ;
#103608=ORIENTED_EDGE ( 'NONE', *, *, #43823, .T. ) ;
#103609=DIRECTION ( 'NONE',  ( 0.000000000000000000, 0.000000000000000000, -1.000000000000000000 ) ) ;
#103610=CIRCLE ( 'NONE', #105659, 0.1000000000000002554 ) ;
#103611=VERTEX_POINT ( 'NONE', #17804 ) ;
#103612=ADVANCED_FACE ( 'NONE', ( #119236 ), #36188, .T. ) ;
#103613=ORIENTED_EDGE ( 'NONE', *, *, #97812, .T. ) ;
#103614=FACE_OUTER_BOUND ( 'NONE', #76438, .T. ) ;
#103615=DIRECTION ( 'NONE',  ( -0.000000000000000000, 1.000000000000000000, -0.000000000000000000 ) ) ;
#103616=CIRCLE ( 'NONE', #128766, 0.1000000000000002554 ) ;
#103617=AXIS2_PLACEMENT_3D ( 'NONE', #74161, #83960, #96352 ) ;
#103618=CARTESIAN_POINT ( 'NONE',  ( -3.550000000000031797, 2.500000000000000000, -6.148780366869526226 ) ) ;
#103619=ORIENTED_EDGE ( 'NONE', *, *, #21654, .F. ) ;
#103620=ORIENTED_EDGE ( 'NONE', *, *, #127743, .F. ) ;
#103621=DIRECTION ( 'NONE',  ( -0.000000000000000000, 1.000000000000000000, -0.000000000000000000 ) ) ;
#103622=DIRECTION ( 'NONE',  ( 0.000000000000000000, 0.000000000000000000, 1.000000000000000000 ) ) ;
#103623=CARTESIAN_POINT ( 'NONE',  ( -2.700000000000031264, 2.500000000000000000, 4.776537180435972196 ) ) ;
#103624=LINE ( 'NONE', #55803, #53443 ) ;
#103625=AXIS2_PLACEMENT_3D ( 'NONE', #109383, #21001, #91037 ) ;
#103626=CARTESIAN_POINT ( 'NONE',  ( -2.950000000000029932, 2.500000000000000000, 2.265063509461097357 ) ) ;
#103627=ORIENTED_EDGE ( 'NONE', *, *, #91612, .T. ) ;
#103628=AXIS2_PLACEMENT_3D ( 'NONE', #21205, #128619, #129262 ) ;
#103630=CIRCLE ( 'NONE', #26263, 0.09999999999999982514 ) ;
#103631=CARTESIAN_POINT ( 'NONE',  ( -3.100000000000028511, 12.50000000000000000, -0.3464101615137782364 ) ) ;
#103632=CARTESIAN_POINT ( 'NONE',  ( 17.49862860983167323, 2.500000000000000000, -4.081131818001370704 ) ) ;
#103633=AXIS2_PLACEMENT_3D ( 'NONE', #114016, #1464, #91790 ) ;
#103634=VECTOR ( 'NONE', #87292, 1000.000000000000000 ) ;
#103635=EDGE_CURVE ( 'NONE', #7958, #94775, #88479, .T. ) ;
#103636=AXIS2_PLACEMENT_3D ( 'NONE', #122464, #9917, #10543 ) ;
#103638=CARTESIAN_POINT ( 'NONE',  ( 2.049999999999948308, 2.500000000000000000, 6.595190528383296780 ) ) ;
#103639=FACE_OUTER_BOUND ( 'NONE', #107729, .T. ) ;
#103640=CARTESIAN_POINT ( 'NONE',  ( 2.949999999999943334, 2.500000000000000000, 6.395190528383296602 ) ) ;
#103641=CARTESIAN_POINT ( 'NONE',  ( 1.249999999999953815, 2.500000000000000000, 1.572243186433545548 ) ) ;
#103642=ORIENTED_EDGE ( 'NONE', *, *, #16995, .F. ) ;
#103643=ADVANCED_FACE ( 'NONE', ( #87829 ), #94646, .T. ) ;
#103644=CARTESIAN_POINT ( 'NONE',  ( 1.849999999999950573, 12.50000000000000000, -1.818653347947326138 ) ) ;
#103645=DIRECTION ( 'NONE',  ( 0.000000000000000000, 0.000000000000000000, 1.000000000000000000 ) ) ;
#103646=DIRECTION ( 'NONE',  ( 0.000000000000000000, 0.000000000000000000, -1.000000000000000000 ) ) ;
#103647=VERTEX_POINT ( 'NONE', #119885 ) ;
#103648=EDGE_CURVE ( 'NONE', #37147, #2544, #71677, .T. ) ;
#103649=EDGE_CURVE ( 'NONE', #105928, #19953, #82148, .T. ) ;
#103650=EDGE_CURVE ( 'NONE', #7926, #62375, #77925, .T. ) ;
#103651=EDGE_CURVE ( 'NONE', #97855, #3084, #110070, .T. ) ;
#103652=CONICAL_SURFACE ( 'NONE', #95327, 0.1000000000000002554, 0.003490658503988666988 ) ;
#103653=CARTESIAN_POINT ( 'NONE',  ( -8.100000000000013856, 12.50000000000000000, -0.3464101615137782364 ) ) ;
#103654=ORIENTED_EDGE ( 'NONE', *, *, #5947, .F. ) ;
#103655=ADVANCED_FACE ( 'NONE', ( #100254 ), #79336, .T. ) ;
#103656=DIRECTION ( 'NONE',  ( -0.000000000000000000, -1.000000000000000000, -0.000000000000000000 ) ) ;
#103657=EDGE_CURVE ( 'NONE', #17700, #15440, #109421, .T. ) ;
#103658=VECTOR ( 'NONE', #111917, 1000.000000000000000 ) ;
#103659=ORIENTED_EDGE ( 'NONE', *, *, #117835, .F. ) ;
#103660=CARTESIAN_POINT ( 'NONE',  ( -7.900000000000011013, 2.500000000000000000, 4.330127018922196314 ) ) ;
#103661=DIRECTION ( 'NONE',  ( -0.000000000000000000, -1.000000000000000000, -0.000000000000000000 ) ) ;
#103662=EDGE_CURVE ( 'NONE', #37879, #35997, #47936, .T. ) ;
#103663=CARTESIAN_POINT ( 'NONE',  ( 4.799999999999937650, 12.50000000000000000, -0.3464101615137782364 ) ) ;
#103664=VECTOR ( 'NONE', #12549, 1000.000000000000000 ) ;
#103665=AXIS2_PLACEMENT_3D ( 'NONE', #36241, #113494, #16563 ) ;
#103666=ORIENTED_EDGE ( 'NONE', *, *, #16686, .F. ) ;
#103667=EDGE_CURVE ( 'NONE', #31864, #71376, #127141, .T. ) ;
#103668=DIRECTION ( 'NONE',  ( 0.000000000000000000, 1.000000000000000000, 0.000000000000000000 ) ) ;
#103669=EDGE_CURVE ( 'NONE', #122087, #25527, #111362, .T. ) ;
#103670=AXIS2_PLACEMENT_3D ( 'NONE', #127658, #17692, #56965 ) ;
#103672=ADVANCED_FACE ( 'NONE', ( #18460 ), #115566, .T. ) ;
#103673=ORIENTED_EDGE ( 'NONE', *, *, #103488, .F. ) ;
#103674=CIRCLE ( 'NONE', #128738, 0.06509327318403745899 ) ;
#103675=EDGE_LOOP ( 'NONE', ( #11720, #63374, #105963, #101135 ) ) ;
#103676=VECTOR ( 'NONE', #87767, 1000.000000000000000 ) ;
#103677=AXIS2_PLACEMENT_3D ( 'NONE', #95329, #83587, #84204 ) ;
#103678=VERTEX_POINT ( 'NONE', #128442 ) ;
#103679=DIRECTION ( 'NONE',  ( 0.000000000000000000, 0.000000000000000000, -1.000000000000000000 ) ) ;
#103680=DIRECTION ( 'NONE',  ( 0.000000000000000000, 1.000000000000000000, 0.000000000000000000 ) ) ;
#103681=FACE_OUTER_BOUND ( 'NONE', #87404, .T. ) ;
#103682=ORIENTED_EDGE ( 'NONE', *, *, #53819, .T. ) ;
#103683=CARTESIAN_POINT ( 'NONE',  ( 0.5999999999999621192, 2.500000000000000000, 0.3464101615137758494 ) ) ;
#103684=DIRECTION ( 'NONE',  ( 0.000000000000000000, 0.000000000000000000, 1.000000000000000000 ) ) ;
#103685=ORIENTED_EDGE ( 'NONE', *, *, #27506, .T. ) ;
#103686=DIRECTION ( 'NONE',  ( 0.000000000000000000, 0.000000000000000000, 1.000000000000000000 ) ) ;
#103687=CONICAL_SURFACE ( 'NONE', #118056, 0.1000000000000000056, 0.003490658503988666988 ) ;
#103688=LINE ( 'NONE', #112858, #124527 ) ;
#103689=CIRCLE ( 'NONE', #122472, 0.06509327318403745899 ) ;
#103690=PLANE ( 'NONE',  #78021 ) ;
#103691=DIRECTION ( 'NONE',  ( 0.000000000000000000, -0.000000000000000000, 1.000000000000000000 ) ) ;
#103692=DIRECTION ( 'NONE',  ( 0.000000000000000000, 1.000000000000000000, 0.000000000000000000 ) ) ;
#103693=DIRECTION ( 'NONE',  ( 0.000000000000000000, -0.000000000000000000, 1.000000000000000000 ) ) ;
#103694=CARTESIAN_POINT ( 'NONE',  ( -8.150000000000012790, 2.500000000000000000, -1.818653347947326138 ) ) ;
#103695=VERTEX_POINT ( 'NONE', #98956 ) ;
#103696=ORIENTED_EDGE ( 'NONE', *, *, #48114, .T. ) ;
#103697=EDGE_LOOP ( 'NONE', ( #74965, #12565, #112248, #31363 ) ) ;
#103698=VERTEX_POINT ( 'NONE', #49235 ) ;
#103699=CARTESIAN_POINT ( 'NONE',  ( 81.97061111377642817, 3.937853021265186548, 6.123961096679600757 ) ) ;
#103700=DIRECTION ( 'NONE',  ( 0.000000000000000000, 0.000000000000000000, 1.000000000000000000 ) ) ;
#103701=PLANE ( 'NONE',  #88646 ) ;
#103702=VERTEX_POINT ( 'NONE', #89134 ) ;
#103703=FACE_BOUND ( 'NONE', #9635, .T. ) ;
#103704=DIRECTION ( 'NONE',  ( -0.000000000000000000, -1.000000000000000000, -0.000000000000000000 ) ) ;
#103705=CARTESIAN_POINT ( 'NONE',  ( 3.949999999999941558, 2.500000000000000000, -1.818653347947326138 ) ) ;
#103706=ADVANCED_FACE ( 'NONE', ( #129091 ), #11108, .T. ) ;
#103707=DIRECTION ( 'NONE',  ( 0.000000000000000000, 0.000000000000000000, 1.000000000000000000 ) ) ;
#103708=CIRCLE ( 'NONE', #18002, 0.1000000000000002554 ) ;
#103709=CARTESIAN_POINT ( 'NONE',  ( 4.999999999999971578, 2.500000000000000000, -2.276824562219559311E-15 ) ) ;
#103710=EDGE_CURVE ( 'NONE', #61453, #28873, #79957, .T. ) ;
#103711=CARTESIAN_POINT ( 'NONE',  ( -7.300000000000016698, 2.500000000000000000, -4.776537180435978414 ) ) ;
#103712=CARTESIAN_POINT ( 'NONE',  ( -11.24999999999996447, 2.500000000000000000, -6.595190528383298556 ) ) ;
#103714=DIRECTION ( 'NONE',  ( 0.000000000000000000, 0.000000000000000000, 1.000000000000000000 ) ) ;
#103715=DIRECTION ( 'NONE',  ( 0.000000000000000000, -0.000000000000000000, 1.000000000000000000 ) ) ;
#103716=DIRECTION ( 'NONE',  ( 0.000000000000000000, 0.000000000000000000, 1.000000000000000000 ) ) ;
#103717=CARTESIAN_POINT ( 'NONE',  ( 4.999999999999936939, 2.500000000000000000, -3.737306695894649700 ) ) ;
#103718=EDGE_CURVE ( 'NONE', #103899, #95311, #78029, .T. ) ;
#103719=CONICAL_SURFACE ( 'NONE', #74755, 0.09999999999999982514, 0.003490658503988666988 ) ;
#103720=AXIS2_PLACEMENT_3D ( 'NONE', #28014, #107856, #16229 ) ;
#103721=ORIENTED_EDGE ( 'NONE', *, *, #69245, .T. ) ;
#103722=ORIENTED_EDGE ( 'NONE', *, *, #16119, .T. ) ;
#103723=ORIENTED_EDGE ( 'NONE', *, *, #10324, .F. ) ;
#103724=VERTEX_POINT ( 'NONE', #100876 ) ;
#103725=ORIENTED_EDGE ( 'NONE', *, *, #48303, .F. ) ;
#103726=EDGE_LOOP ( 'NONE', ( #53045, #92423, #66399, #116698 ) ) ;
#103727=DIRECTION ( 'NONE',  ( 0.000000000000000000, 0.000000000000000000, 1.000000000000000000 ) ) ;
#103728=VERTEX_POINT ( 'NONE', #113277 ) ;
#103729=VERTEX_POINT ( 'NONE', #103469 ) ;
#103730=CIRCLE ( 'NONE', #109977, 0.06509327318403743123 ) ;
#103731=CIRCLE ( 'NONE', #120441, 0.1000000000000000472 ) ;
#103732=CARTESIAN_POINT ( 'NONE',  ( 12.65326442544191998, -1.500000000000190292, 8.428886915957789938 ) ) ;
#103733=DIRECTION ( 'NONE',  ( -0.000000000000000000, 1.000000000000000000, -0.000000000000000000 ) ) ;
#103734=CARTESIAN_POINT ( 'NONE',  ( -10.85000000000000142, 2.500000000000000000, -6.595190528383298556 ) ) ;
#103735=EDGE_LOOP ( 'NONE', ( #56874, #27000, #62982, #107168 ) ) ;
#103736=CARTESIAN_POINT ( 'NONE',  ( -3.150000000000032330, 2.500000000000000000, -6.248780366869526759 ) ) ;
#103737=ORIENTED_EDGE ( 'NONE', *, *, #93369, .T. ) ;
#103738=ORIENTED_EDGE ( 'NONE', *, *, #61463, .F. ) ;
#103739=CARTESIAN_POINT ( 'NONE',  ( 9.149999999999916866, 2.500000000000000000, -1.472243186433550122 ) ) ;
#103740=ORIENTED_EDGE ( 'NONE', *, *, #19265, .T. ) ;
#103741=CARTESIAN_POINT ( 'NONE',  ( 12.49999999999990585, 2.500000000000000000, -5.022947341949754119 ) ) ;
#103742=ORIENTED_EDGE ( 'NONE', *, *, #84427, .F. ) ;
#103743=DIRECTION ( 'NONE',  ( 0.000000000000000000, 0.000000000000000000, 1.000000000000000000 ) ) ;
#103744=CARTESIAN_POINT ( 'NONE',  ( 13.14999999999990088, 12.50000000000000000, 1.883746621131358934 ) ) ;
#103745=FACE_OUTER_BOUND ( 'NONE', #123467, .T. ) ;
#103746=AXIS2_PLACEMENT_3D ( 'NONE', #63184, #92642, #53373 ) ;
#103747=DIRECTION ( 'NONE',  ( -0.000000000000000000, -1.000000000000000000, -0.000000000000000000 ) ) ;
#103748=DIRECTION ( 'NONE',  ( 0.000000000000000000, 0.000000000000000000, 1.000000000000000000 ) ) ;
#103749=CIRCLE ( 'NONE', #80773, 0.1000000000000002554 ) ;
#103750=VECTOR ( 'NONE', #49618, 1000.000000000000000 ) ;
#103751=EDGE_LOOP ( 'NONE', ( #57341, #76290 ) ) ;
#103752=CARTESIAN_POINT ( 'NONE',  ( -8.350000000000008527, 12.50000000000000000, 7.122917578226811486 ) ) ;
#103753=ORIENTED_EDGE ( 'NONE', *, *, #12046, .F. ) ;
#103754=AXIS2_PLACEMENT_3D ( 'NONE', #123001, #83727, #123625 ) ;
#103755=CARTESIAN_POINT ( 'NONE',  ( 17.50000000000000000, 2.500000000000000000, 3.333333333333334370 ) ) ;
#103756=ORIENTED_EDGE ( 'NONE', *, *, #63740, .T. ) ;
#103757=DIRECTION ( 'NONE',  ( -0.000000000000000000, 1.000000000000000000, -0.000000000000000000 ) ) ;
#103758=DIRECTION ( 'NONE',  ( 0.000000000000000000, 0.000000000000000000, 1.000000000000000000 ) ) ;
#103759=EDGE_CURVE ( 'NONE', #48774, #61216, #34125, .T. ) ;
#103760=DIRECTION ( 'NONE',  ( 0.000000000000000000, 0.000000000000000000, -1.000000000000000000 ) ) ;
#103761=EDGE_CURVE ( 'NONE', #17352, #63575, #13162, .T. ) ;
#103762=CARTESIAN_POINT ( 'NONE',  ( 1.049999999999954969, 12.50000000000000000, -6.841600689897077814 ) ) ;
#103763=VERTEX_POINT ( 'NONE', #123110 ) ;
#103764=CIRCLE ( 'NONE', #112079, 0.06509327318403745899 ) ;
#103765=DIRECTION ( 'NONE',  ( 0.000000000000000000, 0.000000000000000000, 1.000000000000000000 ) ) ;
#103766=CONICAL_SURFACE ( 'NONE', #101713, 0.1000000000000002554, 0.003490658503988666988 ) ;
#103767=AXIS2_PLACEMENT_3D ( 'NONE', #41905, #92265, #43200 ) ;
#103768=DIRECTION ( 'NONE',  ( 0.000000000000000000, -0.9999939076577903929, 0.003490651415223739937 ) ) ;
#103769=EDGE_LOOP ( 'NONE', ( #127966, #48217, #108281, #127750 ) ) ;
#103770=VERTEX_POINT ( 'NONE', #61623 ) ;
#103771=EDGE_CURVE ( 'NONE', #53022, #53628, #8965, .T. ) ;
#103772=ORIENTED_EDGE ( 'NONE', *, *, #80756, .F. ) ;
#103773=CARTESIAN_POINT ( 'NONE',  ( -9.550000000000007816, 2.500000000000000000, -6.395190528383296602 ) ) ;
#103774=DIRECTION ( 'NONE',  ( 0.000000000000000000, 0.000000000000000000, 1.000000000000000000 ) ) ;
#103776=LINE ( 'NONE', #101196, #17724 ) ;
#103777=CARTESIAN_POINT ( 'NONE',  ( 16.80072262464530652, 1.717570462274060850, -5.816823748342643263 ) ) ;
#103778=DIRECTION ( 'NONE',  ( -0.000000000000000000, 1.000000000000000000, -0.000000000000000000 ) ) ;
#103779=EDGE_LOOP ( 'NONE', ( #69686, #12256, #91176, #33283 ) ) ;
#103780=CARTESIAN_POINT ( 'NONE',  ( 1.899999999999951283, 12.50000000000000000, 0.3464101615137736845 ) ) ;
#103781=EDGE_CURVE ( 'NONE', #111163, #117766, #65407, .T. ) ;
#103782=EDGE_LOOP ( 'NONE', ( #63614, #958 ) ) ;
#103783=CARTESIAN_POINT ( 'NONE',  ( 0.6499999999999561684, 12.50000000000000000, 2.446380397790835826 ) ) ;
#103784=LINE ( 'NONE', #84784, #3638 ) ;
#103785=CARTESIAN_POINT ( 'NONE',  ( 5.849999999999933920, 12.50000000000000000, -2.230156782645139391 ) ) ;
#103786=DIRECTION ( 'NONE',  ( 0.000000000000000000, -0.9999939076577903929, 0.003490651415223739937 ) ) ;
#103787=EDGE_LOOP ( 'NONE', ( #114948, #92075, #42463, #69737 ) ) ;
#103789=AXIS2_PLACEMENT_3D ( 'NONE', #6505, #28778, #68684 ) ;
#103790=CARTESIAN_POINT ( 'NONE',  ( 10.64999999999990976, 2.500000000000000000, 1.718653347947321386 ) ) ;
#103791=CARTESIAN_POINT ( 'NONE',  ( 10.59999999999990905, 2.500000000000000000, 3.883716857408420431 ) ) ;
#103792=ORIENTED_EDGE ( 'NONE', *, *, #492, .T. ) ;
#103793=ADVANCED_FACE ( 'NONE', ( #121809 ), #60955, .T. ) ;
#103794=ADVANCED_FACE ( 'NONE', ( #81255 ), #52990, .T. ) ;
#103795=EDGE_CURVE ( 'NONE', #52298, #99291, #32077, .T. ) ;
#103796=EDGE_CURVE ( 'NONE', #94042, #10496, #15315, .T. ) ;
#103797=ORIENTED_EDGE ( 'NONE', *, *, #26968, .F. ) ;
#103798=AXIS2_PLACEMENT_3D ( 'NONE', #80625, #81263, #20409 ) ;
#103799=AXIS2_PLACEMENT_3D ( 'NONE', #46201, #88536, #126042 ) ;
#103800=DIRECTION ( 'NONE',  ( 0.000000000000000000, 0.000000000000000000, 1.000000000000000000 ) ) ;
#103801=VERTEX_POINT ( 'NONE', #745 ) ;
#103802=ORIENTED_EDGE ( 'NONE', *, *, #73347, .F. ) ;
#103803=DIRECTION ( 'NONE',  ( 0.000000000000000000, 1.000000000000000000, 0.000000000000000000 ) ) ;
#103804=EDGE_CURVE ( 'NONE', #17144, #114482, #102184, .T. ) ;
#103805=ADVANCED_FACE ( 'NONE', ( #91713 ), #34229, .T. ) ;
#103806=ORIENTED_EDGE ( 'NONE', *, *, #8818, .T. ) ;
#103807=DIRECTION ( 'NONE',  ( -0.000000000000000000, -1.000000000000000000, -0.000000000000000000 ) ) ;
#103808=LINE ( 'NONE', #63881, #46395 ) ;
#103809=VECTOR ( 'NONE', #94, 1000.000000000000000 ) ;
#103810=DIRECTION ( 'NONE',  ( 0.000000000000000000, 0.000000000000000000, 1.000000000000000000 ) ) ;
#103811=VERTEX_POINT ( 'NONE', #63551 ) ;
#103812=EDGE_CURVE ( 'NONE', #89734, #59250, #40496, .T. ) ;
#103813=CIRCLE ( 'NONE', #26458, 0.09999999999999982514 ) ;
#103814=EDGE_CURVE ( 'NONE', #36682, #29463, #42639, .T. ) ;
#103815=DIRECTION ( 'NONE',  ( -4.274815082592931898E-19, -0.9999939076577903929, -0.003490651415223739937 ) ) ;
#103816=DIRECTION ( 'NONE',  ( -0.000000000000000000, 1.000000000000000000, -0.000000000000000000 ) ) ;
#103817=EDGE_LOOP ( 'NONE', ( #27733, #125457 ) ) ;
#103818=CARTESIAN_POINT ( 'NONE',  ( 9.149999999999918643, 12.50000000000000000, 2.165063509461097713 ) ) ;
#103819=EDGE_CURVE ( 'NONE', #78788, #44264, #9072, .T. ) ;
#103820=CARTESIAN_POINT ( 'NONE',  ( 3.549999999999942979, 12.50000000000000000, 1.753560074763284016 ) ) ;
#103821=EDGE_CURVE ( 'NONE', #94166, #118365, #128220, .T. ) ;
#103822=ORIENTED_EDGE ( 'NONE', *, *, #57259, .T. ) ;
#103823=ORIENTED_EDGE ( 'NONE', *, *, #104839, .T. ) ;
#103824=ORIENTED_EDGE ( 'NONE', *, *, #17653, .T. ) ;
#103825=VERTEX_POINT ( 'NONE', #93013 ) ;
#103826=CARTESIAN_POINT ( 'NONE',  ( 9.599999999999917932, 12.50000000000000000, -0.7579135962115916003 ) ) ;
#103827=DIRECTION ( 'NONE',  ( -0.000000000000000000, -1.000000000000000000, -0.000000000000000000 ) ) ;
#103828=FACE_OUTER_BOUND ( 'NONE', #65557, .T. ) ;
#103829=FACE_BOUND ( 'NONE', #23964, .T. ) ;
#103830=ORIENTED_EDGE ( 'NONE', *, *, #72381, .T. ) ;
#103831=CIRCLE ( 'NONE', #95511, 0.09999999999999982514 ) ;
#103833=PLANE ( 'NONE',  #84530 ) ;
#103834=DIRECTION ( 'NONE',  ( -0.000000000000000000, -1.000000000000000000, -0.000000000000000000 ) ) ;
#103835=CONICAL_SURFACE ( 'NONE', #127114, 0.1000000000000002554, 0.003490658503988666988 ) ;
#103836=AXIS2_PLACEMENT_3D ( 'NONE', #85452, #96544, #6865 ) ;
#103837=DIRECTION ( 'NONE',  ( -0.000000000000000000, 1.000000000000000000, -0.000000000000000000 ) ) ;
#103838=CARTESIAN_POINT ( 'NONE',  ( 2.699999999999947331, 12.50000000000000000, -4.676537180435978769 ) ) ;
#103840=AXIS2_PLACEMENT_3D ( 'NONE', #28521, #18036, #96588 ) ;
#103841=AXIS2_PLACEMENT_3D ( 'NONE', #14473, #7724, #53775 ) ;
#103842=LINE ( 'NONE', #14149, #72510 ) ;
#103843=CIRCLE ( 'NONE', #47417, 0.1000000000000002554 ) ;
#103844=EDGE_LOOP ( 'NONE', ( #26362, #72312 ) ) ;
#103845=ORIENTED_EDGE ( 'NONE', *, *, #103067, .F. ) ;
#103846=VERTEX_POINT ( 'NONE', #3333 ) ;
#103847=ORIENTED_EDGE ( 'NONE', *, *, #77926, .F. ) ;
#103848=ORIENTED_EDGE ( 'NONE', *, *, #77593, .F. ) ;
#103849=DIRECTION ( 'NONE',  ( -0.000000000000000000, 1.000000000000000000, -0.000000000000000000 ) ) ;
#103850=CARTESIAN_POINT ( 'NONE',  ( 6.049999999999934097, 12.50000000000000000, -6.148780366869526226 ) ) ;
#103851=AXIS2_PLACEMENT_3D ( 'NONE', #121104, #53019, #82487 ) ;
#103852=ORIENTED_EDGE ( 'NONE', *, *, #104849, .T. ) ;
#103853=FACE_BOUND ( 'NONE', #3119, .T. ) ;
#103854=CIRCLE ( 'NONE', #49493, 0.09999999999999982514 ) ;
#103855=DIRECTION ( 'NONE',  ( 0.000000000000000000, 0.000000000000000000, 1.000000000000000000 ) ) ;
#103856=ADVANCED_FACE ( 'NONE', ( #33455 ), #46736, .T. ) ;
#103857=CONICAL_SURFACE ( 'NONE', #47428, 0.1000000000000000056, 0.003490658503988666988 ) ;
#103858=AXIS2_PLACEMENT_3D ( 'NONE', #81174, #12417, #112574 ) ;
#103859=ADVANCED_FACE ( 'NONE', ( #54361 ), #27947, .T. ) ;
#103860=ORIENTED_EDGE ( 'NONE', *, *, #14812, .F. ) ;
#103861=DIRECTION ( 'NONE',  ( 0.000000000000000000, 1.000000000000000000, 0.000000000000000000 ) ) ;
#103862=FACE_OUTER_BOUND ( 'NONE', #31306, .T. ) ;
#103863=CARTESIAN_POINT ( 'NONE',  ( 9.149999999999920419, 12.50000000000000000, -7.188010851410854052 ) ) ;
#103864=VERTEX_POINT ( 'NONE', #65463 ) ;
#103865=FACE_OUTER_BOUND ( 'NONE', #37981, .T. ) ;
#103866=ORIENTED_EDGE ( 'NONE', *, *, #129554, .T. ) ;
#103867=EDGE_LOOP ( 'NONE', ( #49654, #85071 ) ) ;
#103868=VERTEX_POINT ( 'NONE', #105403 ) ;
#103869=DIRECTION ( 'NONE',  ( -0.000000000000000000, 1.000000000000000000, -0.000000000000000000 ) ) ;
#103870=DIRECTION ( 'NONE',  ( -0.000000000000000000, -1.000000000000000000, -0.000000000000000000 ) ) ;
#103871=CARTESIAN_POINT ( 'NONE',  ( 1.849999999999949685, 2.500000000000000000, -2.511473670974877948 ) ) ;
#103872=EDGE_LOOP ( 'NONE', ( #70983, #128048 ) ) ;
#103873=AXIS2_PLACEMENT_3D ( 'NONE', #20159, #54761, #103879 ) ;
#103874=DIRECTION ( 'NONE',  ( -0.000000000000000000, -1.000000000000000000, -0.000000000000000000 ) ) ;
#103875=LINE ( 'NONE', #14181, #57463 ) ;
#103876=CARTESIAN_POINT ( 'NONE',  ( 13.09999999999990195, 2.500000000000000000, -3.983716857408426293 ) ) ;
#103878=ORIENTED_EDGE ( 'NONE', *, *, #85142, .T. ) ;
#103879=DIRECTION ( 'NONE',  ( 0.000000000000000000, -0.000000000000000000, 1.000000000000000000 ) ) ;
#103880=ORIENTED_EDGE ( 'NONE', *, *, #41797, .T. ) ;
#103881=FACE_OUTER_BOUND ( 'NONE', #52951, .T. ) ;
#103882=AXIS2_PLACEMENT_3D ( 'NONE', #25457, #124973, #74580 ) ;
#103883=ORIENTED_EDGE ( 'NONE', *, *, #100734, .T. ) ;
#103884=CIRCLE ( 'NONE', #24461, 0.06509327318403741736 ) ;
#103885=ORIENTED_EDGE ( 'NONE', *, *, #74940, .F. ) ;
#103886=CARTESIAN_POINT ( 'NONE',  ( -14.34999999999998543, 12.50000000000000000, 2.511473670974877503 ) ) ;
#103887=DIRECTION ( 'NONE',  ( -0.000000000000000000, -1.000000000000000000, -0.000000000000000000 ) ) ;
#103888=PLANE ( 'NONE',  #38399 ) ;
#103889=CARTESIAN_POINT ( 'NONE',  ( -0.4500000000000402012, 2.500000000000000000, 2.265063509461097357 ) ) ;
#103890=CARTESIAN_POINT ( 'NONE',  ( 6.899999999999926636, 2.500000000000000000, -0.2464101615137782308 ) ) ;
#103891=EDGE_LOOP ( 'NONE', ( #124161, #46787, #53132, #71691 ) ) ;
#103892=AXIS2_PLACEMENT_3D ( 'NONE', #12506, #13137, #52435 ) ;
#103893=VECTOR ( 'NONE', #71471, 1000.000000000000000 ) ;
#103894=EDGE_LOOP ( 'NONE', ( #127054, #31121, #48332, #34883 ) ) ;
#103895=ADVANCED_FACE ( 'NONE', ( #96205 ), #61420, .T. ) ;
#103897=CARTESIAN_POINT ( 'NONE',  ( -5.850000000000021849, 12.50000000000000000, -7.188010851410854052 ) ) ;
#103898=CARTESIAN_POINT ( 'NONE',  ( 7.499999999999927169, 2.500000000000000000, -4.922947341949753586 ) ) ;
#103899=VERTEX_POINT ( 'NONE', #26841 ) ;
#103900=ORIENTED_EDGE ( 'NONE', *, *, #31854, .F. ) ;
#103901=DIRECTION ( 'NONE',  ( -0.000000000000000000, 1.000000000000000000, -0.000000000000000000 ) ) ;
#103902=CIRCLE ( 'NONE', #83076, 0.06509327318403745899 ) ;
#103903=AXIS2_PLACEMENT_3D ( 'NONE', #37980, #108007, #126368 ) ;
#103905=DIRECTION ( 'NONE',  ( 0.000000000000000000, 0.000000000000000000, 1.000000000000000000 ) ) ;
#103906=AXIS2_PLACEMENT_3D ( 'NONE', #10763, #70363, #122051 ) ;
#103907=CARTESIAN_POINT ( 'NONE',  ( -7.700000000000016165, 2.500000000000000000, -3.883716857408426648 ) ) ;
#103908=ORIENTED_EDGE ( 'NONE', *, *, #54890, .F. ) ;
#103909=DIRECTION ( 'NONE',  ( 0.000000000000000000, -0.000000000000000000, 1.000000000000000000 ) ) ;
#103910=PLANE ( 'NONE',  #83879 ) ;
#103911=LINE ( 'NONE', #33257, #80263 ) ;
#103913=EDGE_CURVE ( 'NONE', #17273, #88432, #750, .T. ) ;
#103914=DIRECTION ( 'NONE',  ( 0.000000000000000000, 1.000000000000000000, 0.000000000000000000 ) ) ;
#103915=ORIENTED_EDGE ( 'NONE', *, *, #30986, .F. ) ;
#103916=LINE ( 'NONE', #5694, #2755 ) ;
#103917=DIRECTION ( 'NONE',  ( 0.000000000000000000, 1.000000000000000000, 0.000000000000000000 ) ) ;
#103918=ORIENTED_EDGE ( 'NONE', *, *, #51119, .T. ) ;
#103919=ORIENTED_EDGE ( 'NONE', *, *, #66828, .F. ) ;
#103920=EDGE_CURVE ( 'NONE', #45883, #117091, #15710, .T. ) ;
#103922=DIRECTION ( 'NONE',  ( 0.000000000000000000, 1.000000000000000000, 0.000000000000000000 ) ) ;
#103923=CARTESIAN_POINT ( 'NONE',  ( 1.849999999999948130, 2.500000000000000000, 6.148780366869520009 ) ) ;
#103924=AXIS2_PLACEMENT_3D ( 'NONE', #21613, #73929, #121095 ) ;
#103925=DIRECTION ( 'NONE',  ( 0.000000000000000000, 0.000000000000000000, 1.000000000000000000 ) ) ;
#103926=AXIS2_PLACEMENT_3D ( 'NONE', #90491, #81344, #2113 ) ;
#103927=PLANE ( 'NONE',  #46451 ) ;
#103928=CARTESIAN_POINT ( 'NONE',  ( 5.199999999999937117, 12.50000000000000000, -4.676537180435978769 ) ) ;
#103929=AXIS2_PLACEMENT_3D ( 'NONE', #65657, #66303, #64369 ) ;
#103930=DIRECTION ( 'NONE',  ( 0.000000000000000000, -1.000000000000000000, 0.000000000000000000 ) ) ;
#103932=PLANE ( 'NONE',  #125119 ) ;
#103933=DIRECTION ( 'NONE',  ( 0.000000000000000000, 1.000000000000000000, 0.000000000000000000 ) ) ;
#103934=AXIS2_PLACEMENT_3D ( 'NONE', #61857, #14012, #93886 ) ;
#103935=CIRCLE ( 'NONE', #97666, 0.06509327318403745899 ) ;
#103936=DIRECTION ( 'NONE',  ( 0.000000000000000000, 0.000000000000000000, 1.000000000000000000 ) ) ;
#103937=ORIENTED_EDGE ( 'NONE', *, *, #66003, .F. ) ;
#103938=ORIENTED_EDGE ( 'NONE', *, *, #1285, .T. ) ;
#103939=ORIENTED_EDGE ( 'NONE', *, *, #120108, .T. ) ;
#103940=ORIENTED_EDGE ( 'NONE', *, *, #73035, .T. ) ;
#103941=VECTOR ( 'NONE', #12904, 1000.000000000000000 ) ;
#103942=DIRECTION ( 'NONE',  ( 0.000000000000000000, 0.000000000000000000, -1.000000000000000000 ) ) ;
#103943=CARTESIAN_POINT ( 'NONE',  ( 13.74999999999989875, 12.50000000000000000, 1.407149913249508000 ) ) ;
#103944=EDGE_LOOP ( 'NONE', ( #116564, #129044, #116610, #120755 ) ) ;
#103945=DIRECTION ( 'NONE',  ( -0.000000000000000000, -1.000000000000000000, -0.000000000000000000 ) ) ;
#103946=ADVANCED_FACE ( 'NONE', ( #34091 ), #4940, .T. ) ;
#103947=VECTOR ( 'NONE', #117393, 1000.000000000000000 ) ;
#103948=AXIS2_PLACEMENT_3D ( 'NONE', #24668, #11614, #1782 ) ;
#103949=DIRECTION ( 'NONE',  ( 0.000000000000000000, -0.000000000000000000, 1.000000000000000000 ) ) ;
#103950=DIRECTION ( 'NONE',  ( 0.000000000000000000, 0.000000000000000000, -1.000000000000000000 ) ) ;
#103951=EDGE_LOOP ( 'NONE', ( #68209, #31843, #85682, #98509 ) ) ;
#103952=EDGE_CURVE ( 'NONE', #120269, #35997, #78136, .T. ) ;
#103953=DIRECTION ( 'NONE',  ( 0.000000000000000000, -0.9999939076577903929, 0.003490651415223739937 ) ) ;
#103954=ADVANCED_FACE ( 'NONE', ( #86392 ), #103160, .T. ) ;
#103955=DIRECTION ( 'NONE',  ( -0.000000000000000000, -1.000000000000000000, -0.000000000000000000 ) ) ;
#103956=VERTEX_POINT ( 'NONE', #55652 ) ;
#103957=ORIENTED_EDGE ( 'NONE', *, *, #44533, .T. ) ;
#103958=ORIENTED_EDGE ( 'NONE', *, *, #61655, .F. ) ;
#103959=VERTEX_POINT ( 'NONE', #113936 ) ;
#103960=LINE ( 'NONE', #96062, #120079 ) ;
#103961=EDGE_CURVE ( 'NONE', #75979, #126609, #82241, .T. ) ;
#103962=ADVANCED_FACE ( 'NONE', ( #13782 ), #119889, .T. ) ;
#103963=EDGE_CURVE ( 'NONE', #45554, #52604, #94844, .T. ) ;
#103964=AXIS2_PLACEMENT_3D ( 'NONE', #59068, #98985, #6700 ) ;
#103965=EDGE_CURVE ( 'NONE', #7114, #9353, #42545, .T. ) ;
#103966=DIRECTION ( 'NONE',  ( 0.000000000000000000, 1.000000000000000000, 0.000000000000000000 ) ) ;
#103967=DIRECTION ( 'NONE',  ( 0.000000000000000000, -0.000000000000000000, 1.000000000000000000 ) ) ;
#103968=CARTESIAN_POINT ( 'NONE',  ( 4.199999999999939782, 2.500000000000000000, -0.1000000000000022815 ) ) ;
#103969=ORIENTED_EDGE ( 'NONE', *, *, #123421, .T. ) ;
#103970=EDGE_CURVE ( 'NONE', #45836, #60832, #113627, .T. ) ;
#103971=DIRECTION ( 'NONE',  ( 0.000000000000000000, 0.000000000000000000, 1.000000000000000000 ) ) ;
#103972=ORIENTED_EDGE ( 'NONE', *, *, #49808, .T. ) ;
#103973=CARTESIAN_POINT ( 'NONE',  ( -0.2000000000000408673, 12.50000000000000000, -4.048810130592463530 ) ) ;
#103974=CARTESIAN_POINT ( 'NONE',  ( 12.06068301313226598, -2.499999999999744649, -8.632776999392650197 ) ) ;
#103975=LINE ( 'NONE', #83688, #83999 ) ;
#103976=CARTESIAN_POINT ( 'NONE',  ( -5.450000000000023270, 2.500000000000000000, -6.595190528383302109 ) ) ;
#103977=ADVANCED_FACE ( 'NONE', ( #114561 ), #24904, .T. ) ;
#103978=VERTEX_POINT ( 'NONE', #5252 ) ;
#103979=AXIS2_PLACEMENT_3D ( 'NONE', #64603, #114978, #25305 ) ;
#103981=ORIENTED_EDGE ( 'NONE', *, *, #118769, .T. ) ;
#103982=ORIENTED_EDGE ( 'NONE', *, *, #18128, .F. ) ;
#103983=FACE_OUTER_BOUND ( 'NONE', #67680, .T. ) ;
#103984=DIRECTION ( 'NONE',  ( 0.000000000000000000, 0.000000000000000000, -1.000000000000000000 ) ) ;
#103985=LINE ( 'NONE', #83063, #106680 ) ;
#103986=FACE_BOUND ( 'NONE', #68721, .T. ) ;
#103987=DIRECTION ( 'NONE',  ( 0.000000000000000000, -0.9999939076577903929, 0.003490651415223739937 ) ) ;
#103988=DIRECTION ( 'NONE',  ( 0.000000000000000000, -0.9999939076577903929, 0.003490651415223739937 ) ) ;
#103989=CIRCLE ( 'NONE', #66317, 0.1000000000000000472 ) ;
#103990=AXIS2_PLACEMENT_3D ( 'NONE', #124880, #66591, #26677 ) ;
#103991=DIRECTION ( 'NONE',  ( 0.000000000000000000, -0.000000000000000000, 1.000000000000000000 ) ) ;
#103992=CIRCLE ( 'NONE', #81001, 0.09999999999999999167 ) ;
#103994=DIRECTION ( 'NONE',  ( 0.000000000000000000, 0.000000000000000000, 1.000000000000000000 ) ) ;
#103995=DIRECTION ( 'NONE',  ( -0.000000000000000000, -1.000000000000000000, -0.000000000000000000 ) ) ;
#103996=VERTEX_POINT ( 'NONE', #125033 ) ;
#103997=VECTOR ( 'NONE', #101704, 1000.000000000000000 ) ;
#103998=DIRECTION ( 'NONE',  ( 0.000000000000000000, 1.000000000000000000, 0.000000000000000000 ) ) ;
#103999=EDGE_LOOP ( 'NONE', ( #61148, #5986, #11336, #2520 ) ) ;
#104000=ORIENTED_EDGE ( 'NONE', *, *, #66414, .T. ) ;
#104001=ORIENTED_EDGE ( 'NONE', *, *, #73114, .F. ) ;
#104002=EDGE_LOOP ( 'NONE', ( #112897, #89536, #117602, #30081 ) ) ;
#104003=DIRECTION ( 'NONE',  ( 0.000000000000000000, 0.000000000000000000, -1.000000000000000000 ) ) ;
#104004=FACE_BOUND ( 'NONE', #105005, .T. ) ;
#104005=CARTESIAN_POINT ( 'NONE',  ( -8.950000000000009948, 12.50000000000000000, -1.883746621131363597 ) ) ;
#104006=AXIS2_PLACEMENT_3D ( 'NONE', #42215, #122065, #61202 ) ;
#104007=EDGE_CURVE ( 'NONE', #121634, #39004, #121949, .T. ) ;
#104008=AXIS2_PLACEMENT_3D ( 'NONE', #21439, #28207, #68117 ) ;
#104009=ORIENTED_EDGE ( 'NONE', *, *, #94437, .T. ) ;
#104010=CARTESIAN_POINT ( 'NONE',  ( 1.249999999999986899, 2.500000000000000000, 6.395190528383296602 ) ) ;
#104011=PLANE ( 'NONE',  #106289 ) ;
#104012=CIRCLE ( 'NONE', #35071, 0.06509327318403745899 ) ;
#104013=ORIENTED_EDGE ( 'NONE', *, *, #41562, .T. ) ;
#104014=FACE_OUTER_BOUND ( 'NONE', #117019, .T. ) ;
#104015=CIRCLE ( 'NONE', #30875, 0.09999999999999982514 ) ;
#104016=DIRECTION ( 'NONE',  ( 0.000000000000000000, 1.000000000000000000, 0.000000000000000000 ) ) ;
#104017=ADVANCED_FACE ( 'NONE', ( #25529 ), #94749, .T. ) ;
#104018=VECTOR ( 'NONE', #36360, 1000.000000000000000 ) ;
#104019=ORIENTED_EDGE ( 'NONE', *, *, #48959, .F. ) ;
#104020=CARTESIAN_POINT ( 'NONE',  ( -0.4500000000000402012, 12.50000000000000000, 2.099970236277060032 ) ) ;
#104022=AXIS2_PLACEMENT_3D ( 'NONE', #57831, #97741, #8069 ) ;
#104023=CIRCLE ( 'NONE', #26663, 0.06509327318403745899 ) ;
#104024=ORIENTED_EDGE ( 'NONE', *, *, #62616, .F. ) ;
#104025=AXIS2_PLACEMENT_3D ( 'NONE', #106019, #25501, #53693 ) ;
#104026=VECTOR ( 'NONE', #54229, 1000.000000000000000 ) ;
#104027=CARTESIAN_POINT ( 'NONE',  ( -1.450000000000036371, 2.500000000000000000, 2.411473670974873862 ) ) ;
#104028=DIRECTION ( 'NONE',  ( 0.000000000000000000, 1.000000000000000000, 0.000000000000000000 ) ) ;
#104029=CARTESIAN_POINT ( 'NONE',  ( -4.350000000000023626, 2.500000000000000000, 6.048780366869521252 ) ) ;
#104030=ORIENTED_EDGE ( 'NONE', *, *, #26652, .T. ) ;
#104031=VERTEX_POINT ( 'NONE', #98789 ) ;
#104032=CIRCLE ( 'NONE', #70583, 0.1000000000000000472 ) ;
#104033=CARTESIAN_POINT ( 'NONE',  ( 14.19999999999989626, 12.50000000000000000, 0.06509327318403515528 ) ) ;
#104034=ORIENTED_EDGE ( 'NONE', *, *, #3289, .F. ) ;
#104035=DIRECTION ( 'NONE',  ( -0.000000000000000000, -1.000000000000000000, -0.000000000000000000 ) ) ;
#104036=DIRECTION ( 'NONE',  ( 0.000000000000000000, 0.000000000000000000, 1.000000000000000000 ) ) ;
#104037=CIRCLE ( 'NONE', #37149, 0.1000000000000000472 ) ;
#104038=CIRCLE ( 'NONE', #24619, 0.09999999999999982514 ) ;
#104039=EDGE_LOOP ( 'NONE', ( #105023, #52831 ) ) ;
#104040=CARTESIAN_POINT ( 'NONE',  ( -11.05000000000000071, 12.50000000000000000, 2.576566944158910744 ) ) ;
#104042=FACE_OUTER_BOUND ( 'NONE', #62491, .T. ) ;
#104043=DIRECTION ( 'NONE',  ( 0.000000000000000000, 1.000000000000000000, 0.000000000000000000 ) ) ;
#104044=DIRECTION ( 'NONE',  ( 0.000000000000000000, 0.000000000000000000, -1.000000000000000000 ) ) ;
#104045=ORIENTED_EDGE ( 'NONE', *, *, #12843, .F. ) ;
#104046=ADVANCED_FACE ( 'NONE', ( #58250 ), #78541, .T. ) ;
#104047=ORIENTED_EDGE ( 'NONE', *, *, #24616, .T. ) ;
#104048=CARTESIAN_POINT ( 'NONE',  ( 2.299999999999949640, 2.500000000000000000, -4.676537180435977881 ) ) ;
#104049=DIRECTION ( 'NONE',  ( 0.000000000000000000, 1.000000000000000000, 0.000000000000000000 ) ) ;
#104050=DIRECTION ( 'NONE',  ( -4.274815082592931898E-19, -0.9999939076577903929, -0.003490651415223739937 ) ) ;
#104051=ORIENTED_EDGE ( 'NONE', *, *, #101920, .T. ) ;
#104052=ORIENTED_EDGE ( 'NONE', *, *, #128163, .F. ) ;
#104053=ORIENTED_EDGE ( 'NONE', *, *, #115306, .T. ) ;
#104054=DIRECTION ( 'NONE',  ( -0.000000000000000000, -1.000000000000000000, -0.000000000000000000 ) ) ;
#104055=CARTESIAN_POINT ( 'NONE',  ( 9.149999999999916866, 12.50000000000000000, -1.537336459617587581 ) ) ;
#104056=EDGE_CURVE ( 'NONE', #80982, #82263, #107899, .T. ) ;
#104057=CARTESIAN_POINT ( 'NONE',  ( -14.34999999999998543, 2.500000000000000000, -2.511473670974875727 ) ) ;
#104059=LINE ( 'NONE', #14368, #91286 ) ;
#104060=CARTESIAN_POINT ( 'NONE',  ( -12.69999999999999218, 2.500000000000000000, -4.576537180435974683 ) ) ;
#104061=DIRECTION ( 'NONE',  ( 0.000000000000000000, 0.000000000000000000, 1.000000000000000000 ) ) ;
#104062=CARTESIAN_POINT ( 'NONE',  ( -1.700000000000034817, 12.50000000000000000, -4.330127018922201643 ) ) ;
#104063=DIRECTION ( 'NONE',  ( 0.000000000000000000, 0.000000000000000000, -1.000000000000000000 ) ) ;
#104064=EDGE_CURVE ( 'NONE', #86788, #11458, #56917, .T. ) ;
#104065=ADVANCED_FACE ( 'NONE', ( #28785 ), #87679, .T. ) ;
#104066=DIRECTION ( 'NONE',  ( 0.000000000000000000, -0.000000000000000000, 1.000000000000000000 ) ) ;
#104067=VECTOR ( 'NONE', #4698, 1000.000000000000000 ) ;
#104068=VERTEX_POINT ( 'NONE', #37948 ) ;
#104069=AXIS2_PLACEMENT_3D ( 'NONE', #79345, #77396, #117281 ) ;
#104070=ADVANCED_FACE ( 'NONE', ( #99461 ), #69713, .T. ) ;
#104071=CARTESIAN_POINT ( 'NONE',  ( -7.900000000000011013, 2.500000000000000000, 4.230127018922196669 ) ) ;
#104072=ORIENTED_EDGE ( 'NONE', *, *, #128334, .F. ) ;
#104074=ADVANCED_FACE ( 'NONE', ( #9775 ), #48896, .T. ) ;
#104075=DIRECTION ( 'NONE',  ( 0.000000000000000000, 0.000000000000000000, 1.000000000000000000 ) ) ;
#104076=PLANE ( 'NONE',  #42746 ) ;
#104077=CARTESIAN_POINT ( 'NONE',  ( 3.749999999999940492, 2.500000000000000000, 5.802370205355744659 ) ) ;
#104078=AXIS2_PLACEMENT_3D ( 'NONE', #92311, #88614, #2629 ) ;
#104080=CONICAL_SURFACE ( 'NONE', #97810, 0.1000000000000002554, 0.003490658503988666988 ) ;
#104081=CIRCLE ( 'NONE', #26718, 0.06509327318403745899 ) ;
#104082=CARTESIAN_POINT ( 'NONE',  ( 11.64999999999990266, 2.500000000000000000, 2.265063509461097357 ) ) ;
#104083=DIRECTION ( 'NONE',  ( 0.000000000000000000, 1.000000000000000000, 0.000000000000000000 ) ) ;
#104084=CARTESIAN_POINT ( 'NONE',  ( -3.750000000000027534, 2.500000000000000000, 2.757883832488649656 ) ) ;
#104085=ORIENTED_EDGE ( 'NONE', *, *, #118139, .F. ) ;
#104086=DIRECTION ( 'NONE',  ( -0.000000000000000000, 1.000000000000000000, -0.000000000000000000 ) ) ;
#104087=DIRECTION ( 'NONE',  ( 0.000000000000000000, 0.000000000000000000, 1.000000000000000000 ) ) ;
#104088=EDGE_LOOP ( 'NONE', ( #14621, #92711 ) ) ;
#104089=AXIS2_PLACEMENT_3D ( 'NONE', #108683, #45910, #85810 ) ;
#104090=EDGE_LOOP ( 'NONE', ( #4706, #102453, #38444, #81541 ) ) ;
#104091=VERTEX_POINT ( 'NONE', #16970 ) ;
#104092=AXIS2_PLACEMENT_3D ( 'NONE', #39569, #9437, #119372 ) ;
#104093=EDGE_LOOP ( 'NONE', ( #118374, #39353 ) ) ;
#104094=DIRECTION ( 'NONE',  ( -4.274815082592931898E-19, -0.9999939076577903929, -0.003490651415223739937 ) ) ;
#104095=CARTESIAN_POINT ( 'NONE',  ( -11.05000000000000071, 12.50000000000000000, -2.511473670974873951 ) ) ;
#104096=AXIS2_PLACEMENT_3D ( 'NONE', #92377, #25399, #2703 ) ;
#104098=CARTESIAN_POINT ( 'NONE',  ( -10.85000000000000142, 2.500000000000000000, -2.165063509461097713 ) ) ;
#104099=COLOUR_RGB ( '', 0.72549020, 0.75294118, 0.79215686) ;
#104100=DIRECTION ( 'NONE',  ( 0.000000000000000000, 1.000000000000000000, 0.000000000000000000 ) ) ;
#104101=VERTEX_POINT ( 'NONE', #68692 ) ;
#104102=CARTESIAN_POINT ( 'NONE',  ( 87.50000000000001421, -3.975344334345451980, 6.360552532166690476 ) ) ;
#104103=CARTESIAN_POINT ( 'NONE',  ( -6.650000000000019007, 2.500000000000000000, -1.572243186433550211 ) ) ;
#104104=CIRCLE ( 'NONE', #66437, 0.06509327318403745899 ) ;
#104105=ADVANCED_FACE ( 'NONE', ( #98146 ), #47135, .T. ) ;
#104106=DIRECTION ( 'NONE',  ( 0.000000000000000000, 1.000000000000000000, 0.000000000000000000 ) ) ;
#104107=VERTEX_POINT ( 'NONE', #39270 ) ;
#104108=CIRCLE ( 'NONE', #110365, 0.06509327318403745899 ) ;
#104109=VERTEX_POINT ( 'NONE', #129581 ) ;
#104110=ORIENTED_EDGE ( 'NONE', *, *, #58631, .F. ) ;
#104111=EDGE_CURVE ( 'NONE', #114560, #93851, #7086, .T. ) ;
#104112=DIRECTION ( 'NONE',  ( -0.000000000000000000, 1.000000000000000000, -0.000000000000000000 ) ) ;
#104113=EDGE_CURVE ( 'NONE', #7472, #69648, #92807, .T. ) ;
#104114=ADVANCED_FACE ( 'NONE', ( #87039 ), #18935, .T. ) ;
#104115=AXIS2_PLACEMENT_3D ( 'NONE', #69571, #79415, #119311 ) ;
#104116=EDGE_CURVE ( 'NONE', #8586, #94676, #852, .T. ) ;
#104117=DIRECTION ( 'NONE',  ( 0.000000000000000000, 0.000000000000000000, -1.000000000000000000 ) ) ;
#104118=CARTESIAN_POINT ( 'NONE',  ( 13.09999999999989839, 12.50000000000000000, 0.2813168883297361700 ) ) ;
#104119=ADVANCED_FACE ( 'NONE', ( #126978 ), #117913, .T. ) ;
#104120=ORIENTED_EDGE ( 'NONE', *, *, #35668, .T. ) ;
#104121=CARTESIAN_POINT ( 'NONE',  ( 0.8499999999999557909, 2.500000000000000000, -7.288010851410854585 ) ) ;
#104122=CARTESIAN_POINT ( 'NONE',  ( 8.099999999999923261, 2.500000000000000000, -3.883716857408426648 ) ) ;
#104123=AXIS2_PLACEMENT_3D ( 'NONE', #107864, #77745, #39157 ) ;
#104124=CARTESIAN_POINT ( 'NONE',  ( -14.54999999999998472, 2.500000000000000000, -2.165063509461099489 ) ) ;
#104125=CARTESIAN_POINT ( 'NONE',  ( 5.399999999999936406, 2.500000000000000000, -4.922947341949753586 ) ) ;
#104126=ADVANCED_FACE ( 'NONE', ( #107330 ), #17650, .T. ) ;
#104127=CONICAL_SURFACE ( 'NONE', #58174, 0.1000000000000000472, 0.003490658503988666988 ) ;
#104128=AXIS2_PLACEMENT_3D ( 'NONE', #8636, #129110, #18477 ) ;
#104129=EDGE_CURVE ( 'NONE', #2455, #97521, #94947, .T. ) ;
#104130=CARTESIAN_POINT ( 'NONE',  ( -14.14999999999998614, 2.500000000000000000, 2.265063509461101354 ) ) ;
#104131=ORIENTED_EDGE ( 'NONE', *, *, #101863, .T. ) ;
#104132=VERTEX_POINT ( 'NONE', #10415 ) ;
#104134=DIRECTION ( 'NONE',  ( 0.000000000000000000, -0.000000000000000000, 1.000000000000000000 ) ) ;
#104135=DIRECTION ( 'NONE',  ( 0.000000000000000000, 0.000000000000000000, 1.000000000000000000 ) ) ;
#104136=CARTESIAN_POINT ( 'NONE',  ( 3.349999999999942801, 2.500000000000000000, 2.857883832488649301 ) ) ;
#104137=DIRECTION ( 'NONE',  ( 0.000000000000000000, 0.000000000000000000, -1.000000000000000000 ) ) ;
#104138=VERTEX_POINT ( 'NONE', #12971 ) ;
#104139=EDGE_LOOP ( 'NONE', ( #51872, #59009 ) ) ;
#104140=CARTESIAN_POINT ( 'NONE',  ( 9.399999999999915090, 12.50000000000000000, -3.983716857408426293 ) ) ;
#104141=PLANE ( 'NONE',  #107384 ) ;
#104142=DIRECTION ( 'NONE',  ( -0.000000000000000000, 1.000000000000000000, -0.000000000000000000 ) ) ;
#104143=DIRECTION ( 'NONE',  ( -4.274815082592931898E-19, -0.9999939076577903929, -0.003490651415223739937 ) ) ;
#104144=ORIENTED_EDGE ( 'NONE', *, *, #15445, .T. ) ;
#104145=DIRECTION ( 'NONE',  ( 0.000000000000000000, 0.000000000000000000, 1.000000000000000000 ) ) ;
#104146=DIRECTION ( 'NONE',  ( -0.000000000000000000, 1.000000000000000000, -0.000000000000000000 ) ) ;
#104147=CIRCLE ( 'NONE', #87406, 0.1000000000000002554 ) ;
#104148=CONICAL_SURFACE ( 'NONE', #97880, 0.1000000000000002554, 0.003490658503988666988 ) ;
#104149=EDGE_LOOP ( 'NONE', ( #113349, #239, #66507, #38208 ) ) ;
#104150=AXIS2_PLACEMENT_3D ( 'NONE', #121557, #12879, #91462 ) ;
#104151=CARTESIAN_POINT ( 'NONE',  ( -15.79999999999998117, 2.500000000000000000, 0.000000000000000000 ) ) ;
#104152=ORIENTED_EDGE ( 'NONE', *, *, #89063, .F. ) ;
#104153=DIRECTION ( 'NONE',  ( 0.000000000000000000, -0.9999939076577903929, 0.003490651415223739937 ) ) ;
#104154=CONICAL_SURFACE ( 'NONE', #47735, 0.09999999999999982514, 0.003490658503988666988 ) ;
#104155=EDGE_LOOP ( 'NONE', ( #9625, #15375, #124905, #113256 ) ) ;
#104156=DIRECTION ( 'NONE',  ( 0.000000000000000000, 0.000000000000000000, 1.000000000000000000 ) ) ;
#104157=DIRECTION ( 'NONE',  ( 0.000000000000000000, 0.000000000000000000, 1.000000000000000000 ) ) ;
#104158=VERTEX_POINT ( 'NONE', #60814 ) ;
#104159=ORIENTED_EDGE ( 'NONE', *, *, #96119, .T. ) ;
#104161=LINE ( 'NONE', #23029, #62374 ) ;
#104162=VECTOR ( 'NONE', #29295, 1000.000000000000000 ) ;
#104163=CARTESIAN_POINT ( 'NONE',  ( -0.4500000000000402012, 2.500000000000000000, 6.495190528383297135 ) ) ;
#104164=DIRECTION ( 'NONE',  ( 0.000000000000000000, -0.9999939076577903929, 0.003490651415223739937 ) ) ;
#104165=EDGE_CURVE ( 'NONE', #85814, #98726, #25891, .T. ) ;
#104166=VECTOR ( 'NONE', #53065, 1000.000000000000000 ) ;
#104167=LINE ( 'NONE', #95637, #15988 ) ;
#104168=CARTESIAN_POINT ( 'NONE',  ( 3.549999999999941203, 2.500000000000000000, 6.048780366869521252 ) ) ;
#104171=ORIENTED_EDGE ( 'NONE', *, *, #47488, .T. ) ;
#104172=ORIENTED_EDGE ( 'NONE', *, *, #22262, .F. ) ;
#104173=DIRECTION ( 'NONE',  ( -0.000000000000000000, 1.000000000000000000, -0.000000000000000000 ) ) ;
#104174=CARTESIAN_POINT ( 'NONE',  ( -14.59999999999998366, 2.500000000000000000, 0.6928203230275518099 ) ) ;
#104175=CARTESIAN_POINT ( 'NONE',  ( 8.349999999999923261, 2.500000000000000000, -5.902370205355750521 ) ) ;
#104176=AXIS2_PLACEMENT_3D ( 'NONE', #2832, #21848, #42790 ) ;
#104177=CARTESIAN_POINT ( 'NONE',  ( -15.39999999999997904, 2.500000000000000000, -0.6928203230275519209 ) ) ;
#104178=VERTEX_POINT ( 'NONE', #102659 ) ;
#104179=EDGE_LOOP ( 'NONE', ( #91257, #95142, #15087, #105592 ) ) ;
#104180=FACE_BOUND ( 'NONE', #70805, .T. ) ;
#104181=VERTEX_POINT ( 'NONE', #92192 ) ;
#104182=DIRECTION ( 'NONE',  ( 0.000000000000000000, -0.000000000000000000, 1.000000000000000000 ) ) ;
#104183=FACE_OUTER_BOUND ( 'NONE', #72908, .T. ) ;
#104184=VERTEX_POINT ( 'NONE', #51651 ) ;
#104185=FACE_OUTER_BOUND ( 'NONE', #94992, .T. ) ;
#104186=AXIS2_PLACEMENT_3D ( 'NONE', #20217, #556, #3161 ) ;
#104187=CARTESIAN_POINT ( 'NONE',  ( 6.049999999999934097, 12.50000000000000000, 6.148780366869520897 ) ) ;
#104188=DIRECTION ( 'NONE',  ( -4.274815082592931898E-19, -0.9999939076577903929, -0.003490651415223739937 ) ) ;
#104189=DIRECTION ( 'NONE',  ( 0.000000000000000000, -0.000000000000000000, 1.000000000000000000 ) ) ;
#104190=DIRECTION ( 'NONE',  ( 0.000000000000000000, -0.000000000000000000, 1.000000000000000000 ) ) ;
#104191=DIRECTION ( 'NONE',  ( 0.000000000000000000, -0.9999939076577903929, 0.003490651415223739937 ) ) ;
#104192=DIRECTION ( 'NONE',  ( 0.000000000000000000, 0.000000000000000000, 1.000000000000000000 ) ) ;
#104193=LINE ( 'NONE', #15142, #8835 ) ;
#104194=CIRCLE ( 'NONE', #122986, 0.06509327318403741736 ) ;
#104195=DIRECTION ( 'NONE',  ( 0.000000000000000000, 1.000000000000000000, 0.000000000000000000 ) ) ;
#104196=ORIENTED_EDGE ( 'NONE', *, *, #57830, .T. ) ;
#104197=EDGE_LOOP ( 'NONE', ( #4853, #114909 ) ) ;
#104198=VERTEX_POINT ( 'NONE', #83044 ) ;
#104199=DIRECTION ( 'NONE',  ( 0.000000000000000000, 0.000000000000000000, -1.000000000000000000 ) ) ;
#104200=EDGE_LOOP ( 'NONE', ( #7380, #65179, #4578, #5237 ) ) ;
#104201=ORIENTED_EDGE ( 'NONE', *, *, #120186, .F. ) ;
#104202=ORIENTED_EDGE ( 'NONE', *, *, #69970, .T. ) ;
#104203=VERTEX_POINT ( 'NONE', #121653 ) ;
#104204=CIRCLE ( 'NONE', #56264, 0.06509327318403745899 ) ;
#104205=FACE_OUTER_BOUND ( 'NONE', #38289, .T. ) ;
#104206=ADVANCED_FACE ( 'NONE', ( #122959 ), #40592, .T. ) ;
#104207=CARTESIAN_POINT ( 'NONE',  ( 10.84999999999990905, 2.500000000000000000, -6.495190528383302464 ) ) ;
#104209=FACE_OUTER_BOUND ( 'NONE', #13939, .T. ) ;
#104210=CARTESIAN_POINT ( 'NONE',  ( 10.84999999999991260, 12.50000000000000000, -2.099970236277064473 ) ) ;
#104211=DIRECTION ( 'NONE',  ( 0.000000000000000000, 0.000000000000000000, 1.000000000000000000 ) ) ;
#104212=EDGE_CURVE ( 'NONE', #48086, #97670, #2914, .T. ) ;
#104213=ORIENTED_EDGE ( 'NONE', *, *, #113293, .T. ) ;
#104214=EDGE_CURVE ( 'NONE', #28200, #39206, #80278, .T. ) ;
#104215=DIRECTION ( 'NONE',  ( 0.000000000000000000, 1.000000000000000000, 0.000000000000000000 ) ) ;
#104216=ORIENTED_EDGE ( 'NONE', *, *, #96380, .F. ) ;
#104217=AXIS2_PLACEMENT_3D ( 'NONE', #27276, #46945, #105194 ) ;
#104218=AXIS2_PLACEMENT_3D ( 'NONE', #35868, #117609, #58092 ) ;
#104219=EDGE_LOOP ( 'NONE', ( #25969, #92617, #32085, #8894 ) ) ;
#104220=ORIENTED_EDGE ( 'NONE', *, *, #110520, .T. ) ;
#104221=EDGE_CURVE ( 'NONE', #46426, #75204, #11703, .T. ) ;
#104222=DIRECTION ( 'NONE',  ( 0.000000000000000000, 0.000000000000000000, 1.000000000000000000 ) ) ;
#104223=EDGE_CURVE ( 'NONE', #126716, #75929, #23844, .T. ) ;
#104224=ADVANCED_FACE ( 'NONE', ( #60186 ), #111672, .T. ) ;
#104226=ORIENTED_EDGE ( 'NONE', *, *, #90947, .T. ) ;
#104227=EDGE_CURVE ( 'NONE', #106745, #60753, #90736, .T. ) ;
#104228=ADVANCED_FACE ( 'NONE', ( #81727 ), #84478, .T. ) ;
#104229=ORIENTED_EDGE ( 'NONE', *, *, #93414, .T. ) ;
#104232=DIRECTION ( 'NONE',  ( 0.000000000000000000, 1.000000000000000000, 0.000000000000000000 ) ) ;
#104233=DIRECTION ( 'NONE',  ( 0.000000000000000000, 0.000000000000000000, -1.000000000000000000 ) ) ;
#104234=CARTESIAN_POINT ( 'NONE',  ( -8.350000000000010303, 12.50000000000000000, 6.560283801567334372 ) ) ;
#104235=DIRECTION ( 'NONE',  ( -0.000000000000000000, -1.000000000000000000, -0.000000000000000000 ) ) ;
#104236=EDGE_LOOP ( 'NONE', ( #103585, #261, #60123, #80799 ) ) ;
#104237=ADVANCED_FACE ( 'NONE', ( #81110 ), #111569, .T. ) ;
#104238=CARTESIAN_POINT ( 'NONE',  ( -9.350000000000006750, 12.50000000000000000, -2.446380397790840266 ) ) ;
#104239=ORIENTED_EDGE ( 'NONE', *, *, #117671, .T. ) ;
#104240=CIRCLE ( 'NONE', #47814, 0.1000000000000002554 ) ;
#104241=CARTESIAN_POINT ( 'NONE',  ( -13.74999999999998934, 2.500000000000000000, 2.857883832488652853 ) ) ;
#104242=CIRCLE ( 'NONE', #1825, 0.06509327318403745899 ) ;
#104243=ORIENTED_EDGE ( 'NONE', *, *, #37055, .F. ) ;
#104245=CONICAL_SURFACE ( 'NONE', #120965, 0.1000000000000002554, 0.003490658503988666988 ) ;
#104246=ORIENTED_EDGE ( 'NONE', *, *, #15399, .T. ) ;
#104247=VERTEX_POINT ( 'NONE', #40554 ) ;
#104248=CONICAL_SURFACE ( 'NONE', #79130, 0.1000000000000002554, 0.003490658503988666988 ) ;
#104249=CARTESIAN_POINT ( 'NONE',  ( 12.09999999999990195, 12.50000000000000000, -0.7579135962115916003 ) ) ;
#104250=FACE_OUTER_BOUND ( 'NONE', #76860, .T. ) ;
#104251=CIRCLE ( 'NONE', #37456, 0.06509327318403741736 ) ;
#104252=CIRCLE ( 'NONE', #83427, 0.1000000000000002554 ) ;
#104253=AXIS2_PLACEMENT_3D ( 'NONE', #102889, #61041, #71504 ) ;
#104254=DIRECTION ( 'NONE',  ( 0.000000000000000000, 1.000000000000000000, 0.000000000000000000 ) ) ;
#104255=EDGE_LOOP ( 'NONE', ( #51970, #6953, #120030, #108418 ) ) ;
#104257=ORIENTED_EDGE ( 'NONE', *, *, #48643, .F. ) ;
#104258=CARTESIAN_POINT ( 'NONE',  ( -2.300000000000033573, 12.50000000000000000, 4.676537180435972552 ) ) ;
#104259=DIRECTION ( 'NONE',  ( 0.000000000000000000, 1.000000000000000000, 0.000000000000000000 ) ) ;
#104260=DIRECTION ( 'NONE',  ( 0.000000000000000000, 1.000000000000000000, 0.000000000000000000 ) ) ;
#104261=CARTESIAN_POINT ( 'NONE',  ( -1.450000000000035039, 2.500000000000000000, -2.411473670974877859 ) ) ;
#104262=CIRCLE ( 'NONE', #64539, 0.09999999999999982514 ) ;
#104263=DIRECTION ( 'NONE',  ( 0.000000000000000000, 0.000000000000000000, 1.000000000000000000 ) ) ;
#104264=CIRCLE ( 'NONE', #8108, 0.06509327318403745899 ) ;
#104265=ORIENTED_EDGE ( 'NONE', *, *, #61544, .F. ) ;
#104266=EDGE_CURVE ( 'NONE', #86566, #50747, #38435, .T. ) ;
#104267=ADVANCED_FACE ( 'NONE', ( #100719 ), #111854, .T. ) ;
#104268=ORIENTED_EDGE ( 'NONE', *, *, #87093, .T. ) ;
#104269=CARTESIAN_POINT ( 'NONE',  ( 12.49999999999993960, 2.500000000000000000, -4.330127018922201643 ) ) ;
#104270=CARTESIAN_POINT ( 'NONE',  ( 17.50000000000000000, 2.500000000000000888, -4.040567763475094942 ) ) ;
#104271=VECTOR ( 'NONE', #85981, 1000.000000000000000 ) ;
#104272=ADVANCED_FACE ( 'NONE', ( #102029 ), #34319, .T. ) ;
#104273=CONICAL_SURFACE ( 'NONE', #129345, 0.1000000000000002554, 0.003490658503988666988 ) ;
#104276=CARTESIAN_POINT ( 'NONE',  ( 3.349999999999943689, 2.500000000000000000, 1.572243186433545548 ) ) ;
#104277=EDGE_CURVE ( 'NONE', #112874, #35339, #59369, .T. ) ;
#104278=LINE ( 'NONE', #82723, #106627 ) ;
#104279=LINE ( 'NONE', #64349, #74733 ) ;
#104280=ORIENTED_EDGE ( 'NONE', *, *, #67226, .F. ) ;
#104281=ADVANCED_FACE ( 'NONE', ( #80470 ), #19638, .T. ) ;
#104282=EDGE_CURVE ( 'NONE', #70210, #115346, #17556, .T. ) ;
#104283=CARTESIAN_POINT ( 'NONE',  ( 4.349999999999936584, 2.500000000000000000, 6.148780366869520009 ) ) ;
#104284=EDGE_CURVE ( 'NONE', #56443, #28355, #104593, .T. ) ;
#104285=DIRECTION ( 'NONE',  ( -4.274815082592931898E-19, -0.9999939076577903929, -0.003490651415223739937 ) ) ;
#104287=CIRCLE ( 'NONE', #64561, 0.06509327318403745899 ) ;
#104288=EDGE_LOOP ( 'NONE', ( #55565, #25851 ) ) ;
#104289=AXIS2_PLACEMENT_3D ( 'NONE', #6165, #107608, #27115 ) ;
#104290=EDGE_CURVE ( 'NONE', #82143, #15440, #69809, .T. ) ;
#104292=AXIS2_PLACEMENT_3D ( 'NONE', #103164, #123440, #82894 ) ;
#104294=DIRECTION ( 'NONE',  ( 0.000000000000000000, 0.000000000000000000, 1.000000000000000000 ) ) ;
#104295=ORIENTED_EDGE ( 'NONE', *, *, #74977, .T. ) ;
#104296=CARTESIAN_POINT ( 'NONE',  ( 8.749999999999918288, 2.500000000000000000, -1.472243186433550122 ) ) ;
#104297=AXIS2_PLACEMENT_3D ( 'NONE', #104364, #114816, #112901 ) ;
#104298=FACE_OUTER_BOUND ( 'NONE', #62208, .T. ) ;
#104299=CARTESIAN_POINT ( 'NONE',  ( -2.700000000000031264, 2.500000000000000000, 4.576537180435972019 ) ) ;
#104300=ORIENTED_EDGE ( 'NONE', *, *, #82968, .T. ) ;
#104301=CARTESIAN_POINT ( 'NONE',  ( 6.649999999999930189, 2.500000000000000000, -2.957883832488653830 ) ) ;
#104302=CONICAL_SURFACE ( 'NONE', #108496, 0.1000000000000000472, 0.003490658503988666988 ) ;
#104303=CARTESIAN_POINT ( 'NONE',  ( -7.500000000000013323, 12.50000000000000000, 5.022947341949748790 ) ) ;
#104304=AXIS2_PLACEMENT_3D ( 'NONE', #7566, #48813, #67784 ) ;
#104305=EDGE_CURVE ( 'NONE', #35339, #112874, #107458, .T. ) ;
#104306=VERTEX_POINT ( 'NONE', #95429 ) ;
#104307=DIRECTION ( 'NONE',  ( 0.000000000000000000, 0.000000000000000000, -1.000000000000000000 ) ) ;
#104308=VECTOR ( 'NONE', #55471, 1000.000000000000000 ) ;
#104309=ORIENTED_EDGE ( 'NONE', *, *, #63174, .T. ) ;
#104310=ORIENTED_EDGE ( 'NONE', *, *, #111890, .F. ) ;
#104311=DIRECTION ( 'NONE',  ( 0.000000000000000000, -0.000000000000000000, 1.000000000000000000 ) ) ;
#104312=DIRECTION ( 'NONE',  ( -0.000000000000000000, 1.000000000000000000, -0.000000000000000000 ) ) ;
#104313=FACE_OUTER_BOUND ( 'NONE', #88827, .T. ) ;
#104314=VERTEX_POINT ( 'NONE', #105887 ) ;
#104315=DIRECTION ( 'NONE',  ( 0.000000000000000000, 0.000000000000000000, -1.000000000000000000 ) ) ;
#104316=LINE ( 'NONE', #101743, #29379 ) ;
#104317=ORIENTED_EDGE ( 'NONE', *, *, #115589, .T. ) ;
#104318=CARTESIAN_POINT ( 'NONE',  ( -9.400000000000007461, 2.500000000000000000, 3.983716857408420076 ) ) ;
#104319=PLANE ( 'NONE',  #126575 ) ;
#104320=EDGE_CURVE ( 'NONE', #44872, #8732, #123582, .T. ) ;
#104321=CARTESIAN_POINT ( 'NONE',  ( -0.6000000000000323963, 2.500000000000000000, 0.3464101615137759604 ) ) ;
#104323=VECTOR ( 'NONE', #86938, 1000.000000000000000 ) ;
#104325=DIRECTION ( 'NONE',  ( 0.000000000000000000, -0.9999939076577903929, 0.003490651415223739937 ) ) ;
#104326=CARTESIAN_POINT ( 'NONE',  ( 8.349999999999919709, 12.50000000000000000, 7.188010851410848723 ) ) ;
#104327=CONICAL_SURFACE ( 'NONE', #98061, 0.09999999999999982514, 0.003490658503988666988 ) ;
#104328=ORIENTED_EDGE ( 'NONE', *, *, #61643, .F. ) ;
#104329=EDGE_LOOP ( 'NONE', ( #190, #30033 ) ) ;
#104330=VERTEX_POINT ( 'NONE', #115044 ) ;
#104331=VERTEX_POINT ( 'NONE', #16196 ) ;
#104332=CARTESIAN_POINT ( 'NONE',  ( -8.950000000000011724, 12.50000000000000000, -6.148780366869520897 ) ) ;
#104333=FACE_OUTER_BOUND ( 'NONE', #74391, .T. ) ;
#104334=FACE_OUTER_BOUND ( 'NONE', #62053, .T. ) ;
#104335=VERTEX_POINT ( 'NONE', #24111 ) ;
#104336=EDGE_CURVE ( 'NONE', #107226, #55968, #30118, .T. ) ;
#104337=FACE_BOUND ( 'NONE', #58627, .T. ) ;
#104338=CARTESIAN_POINT ( 'NONE',  ( -9.550000000000002487, 2.500000000000000000, 6.595190528383296780 ) ) ;
#104339=CARTESIAN_POINT ( 'NONE',  ( -5.400000000000023448, 2.500000000000000000, -4.922947341949753586 ) ) ;
#104340=AXIS2_PLACEMENT_3D ( 'NONE', #8135, #15365, #115502 ) ;
#104341=CONICAL_SURFACE ( 'NONE', #83517, 0.1000000000000002554, 0.003490658503988666988 ) ;
#104342=LINE ( 'NONE', #122692, #65873 ) ;
#104343=CONICAL_SURFACE ( 'NONE', #60543, 0.1000000000000000472, 0.003490658503988666988 ) ;
#104344=DIRECTION ( 'NONE',  ( 0.000000000000000000, -0.9999939076577903929, 0.003490651415223739937 ) ) ;
#104345=DIRECTION ( 'NONE',  ( 0.000000000000000000, 1.000000000000000000, 0.000000000000000000 ) ) ;
#104346=DIRECTION ( 'NONE',  ( 0.000000000000000000, 0.000000000000000000, 1.000000000000000000 ) ) ;
#104347=DIRECTION ( 'NONE',  ( -4.274815082592931898E-19, -0.9999939076577903929, -0.003490651415223739937 ) ) ;
#104348=DIRECTION ( 'NONE',  ( 0.000000000000000000, 0.000000000000000000, 1.000000000000000000 ) ) ;
#104349=CARTESIAN_POINT ( 'NONE',  ( -10.65000000000000213, 2.500000000000000000, 6.148780366869520009 ) ) ;
#104350=AXIS2_PLACEMENT_3D ( 'NONE', #100444, #103680, #72919 ) ;
#104351=DIRECTION ( 'NONE',  ( -0.000000000000000000, 1.000000000000000000, -0.000000000000000000 ) ) ;
#104352=AXIS2_PLACEMENT_3D ( 'NONE', #105226, #84296, #17967 ) ;
#104353=ORIENTED_EDGE ( 'NONE', *, *, #117782, .F. ) ;
#104354=ORIENTED_EDGE ( 'NONE', *, *, #54890, .T. ) ;
#104355=ORIENTED_EDGE ( 'NONE', *, *, #27251, .T. ) ;
#104356=ORIENTED_EDGE ( 'NONE', *, *, #66156, .T. ) ;
#104357=DIRECTION ( 'NONE',  ( 0.000000000000000000, 0.000000000000000000, 1.000000000000000000 ) ) ;
#104358=VERTEX_POINT ( 'NONE', #103319 ) ;
#104359=CARTESIAN_POINT ( 'NONE',  ( 12.29999999999990656, 12.50000000000000000, 3.983716857408420964 ) ) ;
#104360=VERTEX_POINT ( 'NONE', #73850 ) ;
#104361=ORIENTED_EDGE ( 'NONE', *, *, #7739, .T. ) ;
#104362=EDGE_CURVE ( 'NONE', #96862, #78573, #124887, .T. ) ;
#104363=CARTESIAN_POINT ( 'NONE',  ( 8.512291507236847465, -2.500000000000381473, 9.502944100472593192 ) ) ;
#104364=CARTESIAN_POINT ( 'NONE',  ( -3.950000000000024603, 12.50000000000000000, 1.818653347947321475 ) ) ;
#104365=CARTESIAN_POINT ( 'NONE',  ( -5.850000000000021849, 2.500000000000000000, -1.572243186433550211 ) ) ;
#104366=AXIS2_PLACEMENT_3D ( 'NONE', #109742, #60017, #99924 ) ;
#104367=CARTESIAN_POINT ( 'NONE',  ( -14.34999999999998543, 2.500000000000000000, -2.511473670974875727 ) ) ;
#104368=ORIENTED_EDGE ( 'NONE', *, *, #106521, .T. ) ;
#104369=EDGE_CURVE ( 'NONE', #83004, #107108, #94132, .T. ) ;
#104370=ORIENTED_EDGE ( 'NONE', *, *, #85301, .T. ) ;
#104371=EDGE_LOOP ( 'NONE', ( #36807, #44261, #69171, #17800 ) ) ;
#104372=DIRECTION ( 'NONE',  ( 0.000000000000000000, 0.000000000000000000, 1.000000000000000000 ) ) ;
#104373=ORIENTED_EDGE ( 'NONE', *, *, #68733, .F. ) ;
#104374=ADVANCED_FACE ( 'NONE', ( #35234 ), #53573, .T. ) ;
#104376=EDGE_CURVE ( 'NONE', #75521, #122569, #56131, .T. ) ;
#104377=EDGE_CURVE ( 'NONE', #127091, #38693, #103960, .T. ) ;
#104378=VERTEX_POINT ( 'NONE', #5096 ) ;
#104379=EDGE_CURVE ( 'NONE', #107914, #47637, #59459, .T. ) ;
#104380=ORIENTED_EDGE ( 'NONE', *, *, #43160, .F. ) ;
#104381=CIRCLE ( 'NONE', #121100, 0.06509327318403741736 ) ;
#104382=DIRECTION ( 'NONE',  ( 0.000000000000000000, 0.000000000000000000, 1.000000000000000000 ) ) ;
#104383=DIRECTION ( 'NONE',  ( -0.000000000000000000, -1.000000000000000000, -0.000000000000000000 ) ) ;
#104384=CARTESIAN_POINT ( 'NONE',  ( -8.950000000000009948, 12.50000000000000000, -6.776507416713035248 ) ) ;
#104385=DIRECTION ( 'NONE',  ( 0.000000000000000000, -0.000000000000000000, 1.000000000000000000 ) ) ;
#104386=DIRECTION ( 'NONE',  ( 0.000000000000000000, 0.000000000000000000, -1.000000000000000000 ) ) ;
#104387=VECTOR ( 'NONE', #58511, 1000.000000000000000 ) ;
#104388=EDGE_CURVE ( 'NONE', #60541, #113663, #82440, .T. ) ;
#104389=EDGE_LOOP ( 'NONE', ( #79589, #88514, #17484, #79745 ) ) ;
#104390=CARTESIAN_POINT ( 'NONE',  ( -9.600000000000006750, 2.500000000000000000, 5.022947341949748790 ) ) ;
#104392=EDGE_CURVE ( 'NONE', #84812, #116290, #9261, .T. ) ;
#104393=EDGE_LOOP ( 'NONE', ( #19688, #105402 ) ) ;
#104394=CARTESIAN_POINT ( 'NONE',  ( 17.50000000000000000, 2.499999999999999556, 0.3333333333333366455 ) ) ;
#104395=AXIS2_PLACEMENT_3D ( 'NONE', #10250, #122155, #90742 ) ;
#104396=CIRCLE ( 'NONE', #33311, 0.09999999999999982514 ) ;
#104397=ORIENTED_EDGE ( 'NONE', *, *, #112829, .T. ) ;
#104398=CARTESIAN_POINT ( 'NONE',  ( 3.099999999999945466, 2.500000000000000000, 0.3464101615137735735 ) ) ;
#104399=DIRECTION ( 'NONE',  ( 0.000000000000000000, 1.000000000000000000, 0.000000000000000000 ) ) ;
#104400=VECTOR ( 'NONE', #113510, 1000.000000000000000 ) ;
#104401=FACE_OUTER_BOUND ( 'NONE', #61231, .T. ) ;
#104402=CARTESIAN_POINT ( 'NONE',  ( 4.799999999999939426, 2.500000000000000000, -4.576537180435977348 ) ) ;
#104403=EDGE_LOOP ( 'NONE', ( #24927, #107246 ) ) ;
#104404=DIRECTION ( 'NONE',  ( 0.000000000000000000, 0.000000000000000000, 1.000000000000000000 ) ) ;
#104405=VECTOR ( 'NONE', #110720, 1000.000000000000000 ) ;
#104406=CARTESIAN_POINT ( 'NONE',  ( -8.750000000000005329, 12.50000000000000000, 5.867463478539781896 ) ) ;
#104407=ORIENTED_EDGE ( 'NONE', *, *, #1288, .T. ) ;
#104408=ORIENTED_EDGE ( 'NONE', *, *, #68155, .T. ) ;
#104409=ORIENTED_EDGE ( 'NONE', *, *, #27220, .T. ) ;
#104410=CARTESIAN_POINT ( 'NONE',  ( 4.999999999999935163, 12.50000000000000000, 0.6277270498435120194 ) ) ;
#104411=DIRECTION ( 'NONE',  ( -0.000000000000000000, 1.000000000000000000, -0.000000000000000000 ) ) ;
#104413=CARTESIAN_POINT ( 'NONE',  ( -8.150000000000009237, 2.500000000000000000, 6.048780366869520364 ) ) ;
#104414=DIRECTION ( 'NONE',  ( 0.000000000000000000, 0.000000000000000000, 1.000000000000000000 ) ) ;
#104415=DIRECTION ( 'NONE',  ( 0.000000000000000000, 1.000000000000000000, 0.000000000000000000 ) ) ;
#104416=AXIS2_PLACEMENT_3D ( 'NONE', #44788, #123967, #34333 ) ;
#104417=ORIENTED_EDGE ( 'NONE', *, *, #84108, .T. ) ;
#104418=PLANE ( 'NONE',  #111221 ) ;
#104419=CONICAL_SURFACE ( 'NONE', #70971, 0.1000000000000002554, 0.003490658503988666988 ) ;
#104420=AXIS2_PLACEMENT_3D ( 'NONE', #35205, #75117, #105214 ) ;
#104421=ORIENTED_EDGE ( 'NONE', *, *, #68445, .T. ) ;
#104422=CARTESIAN_POINT ( 'NONE',  ( -13.29999999999999005, 12.50000000000000000, -4.265033745738161741 ) ) ;
#104423=DIRECTION ( 'NONE',  ( 0.000000000000000000, -0.000000000000000000, 1.000000000000000000 ) ) ;
#104424=EDGE_CURVE ( 'NONE', #69263, #4103, #103055, .T. ) ;
#104425=CARTESIAN_POINT ( 'NONE',  ( 7.099999999999928590, 2.500000000000000000, -4.230127018922201998 ) ) ;
#104426=AXIS2_PLACEMENT_3D ( 'NONE', #97015, #16504, #7980 ) ;
#104427=ORIENTED_EDGE ( 'NONE', *, *, #18414, .T. ) ;
#104428=AXIS2_PLACEMENT_3D ( 'NONE', #40993, #101181, #19375 ) ;
#104429=EDGE_CURVE ( 'NONE', #8018, #33146, #46313, .T. ) ;
#104430=CIRCLE ( 'NONE', #14532, 0.06509327318403745899 ) ;
#104431=EDGE_CURVE ( 'NONE', #46303, #117313, #42440, .T. ) ;
#104432=CARTESIAN_POINT ( 'NONE',  ( -4.400000000000025224, 2.500000000000000000, 4.776537180435972196 ) ) ;
#104433=DIRECTION ( 'NONE',  ( 0.000000000000000000, 0.000000000000000000, 1.000000000000000000 ) ) ;
#104434=CONICAL_SURFACE ( 'NONE', #50086, 0.1000000000000000056, 0.003490658503988666988 ) ;
#104435=EDGE_LOOP ( 'NONE', ( #30236, #100253 ) ) ;
#104436=ADVANCED_FACE ( 'NONE', ( #48917 ), #69166, .T. ) ;
#104437=CARTESIAN_POINT ( 'NONE',  ( -9.150000000000009237, 2.500000000000000000, -2.165063509461101710 ) ) ;
#104438=VECTOR ( 'NONE', #121325, 1000.000000000000000 ) ;
#104439=AXIS2_PLACEMENT_3D ( 'NONE', #25724, #15240, #85921 ) ;
#104440=ORIENTED_EDGE ( 'NONE', *, *, #27105, .T. ) ;
#104441=EDGE_LOOP ( 'NONE', ( #99467, #34444 ) ) ;
#104442=CARTESIAN_POINT ( 'NONE',  ( 4.599999999999940137, 2.500000000000000000, -4.430127018922202176 ) ) ;
#104443=ORIENTED_EDGE ( 'NONE', *, *, #97078, .F. ) ;
#104444=CARTESIAN_POINT ( 'NONE',  ( -10.40000000000000213, 12.50000000000000000, -0.06509327318403970719 ) ) ;
#104446=CARTESIAN_POINT ( 'NONE',  ( -7.050000000000013145, 2.500000000000000000, 2.265063509461097357 ) ) ;
#104447=ORIENTED_EDGE ( 'NONE', *, *, #84580, .T. ) ;
#104448=FACE_BOUND ( 'NONE', #116955, .T. ) ;
#104449=DIRECTION ( 'NONE',  ( 0.000000000000000000, 0.000000000000000000, -1.000000000000000000 ) ) ;
#104450=CARTESIAN_POINT ( 'NONE',  ( 10.44999999999991047, 2.500000000000000000, -6.595190528383302109 ) ) ;
#104451=EDGE_LOOP ( 'NONE', ( #98911, #41148 ) ) ;
#104452=DIRECTION ( 'NONE',  ( 0.000000000000000000, -0.9999939076577903929, 0.003490651415223739937 ) ) ;
#104453=DIRECTION ( 'NONE',  ( 0.000000000000000000, 0.000000000000000000, 1.000000000000000000 ) ) ;
#104454=EDGE_CURVE ( 'NONE', #49071, #43610, #80082, .T. ) ;
#104455=ORIENTED_EDGE ( 'NONE', *, *, #8992, .T. ) ;
#104456=ORIENTED_EDGE ( 'NONE', *, *, #109419, .T. ) ;
#104457=ORIENTED_EDGE ( 'NONE', *, *, #101847, .T. ) ;
#104458=FACE_OUTER_BOUND ( 'NONE', #31423, .T. ) ;
#104459=CARTESIAN_POINT ( 'NONE',  ( -9.800000000000006040, 2.500000000000000000, 0.3464101615137735735 ) ) ;
#104461=DIRECTION ( 'NONE',  ( -0.000000000000000000, -1.000000000000000000, -0.000000000000000000 ) ) ;
#104462=FACE_BOUND ( 'NONE', #67086, .T. ) ;
#104463=VERTEX_POINT ( 'NONE', #107818 ) ;
#104465=DIRECTION ( 'NONE',  ( 0.000000000000000000, 1.000000000000000000, 0.000000000000000000 ) ) ;
#104466=CARTESIAN_POINT ( 'NONE',  ( 7.299999999999924327, 12.50000000000000000, 0.3464101615137735735 ) ) ;
#104467=CARTESIAN_POINT ( 'NONE',  ( 6.649999999999929301, 2.500000000000000000, -2.165063509461101710 ) ) ;
#104468=ADVANCED_FACE ( 'NONE', ( #27307 ), #105406, .T. ) ;
#104469=CARTESIAN_POINT ( 'NONE',  ( -9.150000000000009237, 12.50000000000000000, 1.407149913249508000 ) ) ;
#104471=CONICAL_SURFACE ( 'NONE', #62730, 0.1000000000000000472, 0.003490658503988666988 ) ;
#104472=CARTESIAN_POINT ( 'NONE',  ( 0.1999999999999627909, 12.50000000000000000, 0.3464101615137758494 ) ) ;
#104473=LINE ( 'NONE', #33804, #55770 ) ;
#104474=VECTOR ( 'NONE', #76266, 1000.000000000000000 ) ;
#104475=CONICAL_SURFACE ( 'NONE', #18792, 0.09999999999999999167, 0.003490658503988666988 ) ;
#104476=ORIENTED_EDGE ( 'NONE', *, *, #92553, .F. ) ;
#104477=ORIENTED_EDGE ( 'NONE', *, *, #44710, .T. ) ;
#104478=ORIENTED_EDGE ( 'NONE', *, *, #21917, .T. ) ;
#104479=ORIENTED_EDGE ( 'NONE', *, *, #74846, .T. ) ;
#104480=ORIENTED_EDGE ( 'NONE', *, *, #14633, .T. ) ;
#104481=DIRECTION ( 'NONE',  ( 0.000000000000000000, 0.000000000000000000, 1.000000000000000000 ) ) ;
#104483=FACE_OUTER_BOUND ( 'NONE', #32912, .T. ) ;
#104484=ORIENTED_EDGE ( 'NONE', *, *, #19997, .T. ) ;
#104485=EDGE_CURVE ( 'NONE', #120320, #27458, #66601, .T. ) ;
#104486=FACE_BOUND ( 'NONE', #100105, .T. ) ;
#104487=DIRECTION ( 'NONE',  ( 0.000000000000000000, 1.000000000000000000, 0.000000000000000000 ) ) ;
#104488=AXIS2_PLACEMENT_3D ( 'NONE', #48436, #119112, #16999 ) ;
#104489=DIRECTION ( 'NONE',  ( 0.000000000000000000, 0.000000000000000000, -1.000000000000000000 ) ) ;
#104490=ORIENTED_EDGE ( 'NONE', *, *, #20346, .F. ) ;
#104491=CARTESIAN_POINT ( 'NONE',  ( -13.29999999999999005, 2.500000000000000000, 0.1000000000000018513 ) ) ;
#104492=EDGE_CURVE ( 'NONE', #75483, #24119, #19424, .T. ) ;
#104493=DIRECTION ( 'NONE',  ( -0.000000000000000000, 1.000000000000000000, -0.000000000000000000 ) ) ;
#104494=DIRECTION ( 'NONE',  ( 0.000000000000000000, 1.000000000000000000, 0.000000000000000000 ) ) ;
#104495=ORIENTED_EDGE ( 'NONE', *, *, #55306, .T. ) ;
#104496=LINE ( 'NONE', #5640, #47146 ) ;
#104497=ORIENTED_EDGE ( 'NONE', *, *, #114602, .T. ) ;
#104498=ORIENTED_EDGE ( 'NONE', *, *, #18913, .T. ) ;
#104500=PLANE ( 'NONE',  #115345 ) ;
#104501=CARTESIAN_POINT ( 'NONE',  ( 0.1999999999999627909, 2.500000000000000000, 0.3464101615137758494 ) ) ;
#104502=CARTESIAN_POINT ( 'NONE',  ( -15.19999999999998330, 2.500000000000000000, 0.2464101615137758439 ) ) ;
#104503=ORIENTED_EDGE ( 'NONE', *, *, #43299, .T. ) ;
#104504=CARTESIAN_POINT ( 'NONE',  ( -10.65000000000000391, 2.500000000000000000, -1.818653347947322141 ) ) ;
#104505=AXIS2_PLACEMENT_3D ( 'NONE', #80564, #50, #91021 ) ;
#104506=DIRECTION ( 'NONE',  ( 0.000000000000000000, 0.000000000000000000, 1.000000000000000000 ) ) ;
#104507=AXIS2_PLACEMENT_3D ( 'NONE', #15946, #95820, #125906 ) ;
#104508=EDGE_CURVE ( 'NONE', #51768, #29710, #9618, .T. ) ;
#104509=CARTESIAN_POINT ( 'NONE',  ( -2.900000000000029221, 2.500000000000000000, -0.5928203230275541635 ) ) ;
#104511=DIRECTION ( 'NONE',  ( 0.000000000000000000, 1.000000000000000000, 0.000000000000000000 ) ) ;
#104512=ORIENTED_EDGE ( 'NONE', *, *, #36889, .F. ) ;
#104513=FACE_OUTER_BOUND ( 'NONE', #103817, .T. ) ;
#104514=VERTEX_POINT ( 'NONE', #48252 ) ;
#104515=DIRECTION ( 'NONE',  ( -0.000000000000000000, -1.000000000000000000, -0.000000000000000000 ) ) ;
#104516=CIRCLE ( 'NONE', #48097, 0.1000000000000000472 ) ;
#104517=ADVANCED_FACE ( 'NONE', ( #126172 ), #116975, .T. ) ;
#104518=ORIENTED_EDGE ( 'NONE', *, *, #43503, .T. ) ;
#104519=ORIENTED_EDGE ( 'NONE', *, *, #40246, .F. ) ;
#104520=DIRECTION ( 'NONE',  ( -0.000000000000000000, 1.000000000000000000, -0.000000000000000000 ) ) ;
#104521=CARTESIAN_POINT ( 'NONE',  ( 11.04999999999991012, 2.500000000000000000, 6.841600689897072485 ) ) ;
#104522=ADVANCED_FACE ( 'NONE', ( #58725 ), #23638, .T. ) ;
#104523=DIRECTION ( 'NONE',  ( -4.274815082592931898E-19, -0.9999939076577903929, -0.003490651415223739937 ) ) ;
#104524=LINE ( 'NONE', #124823, #42550 ) ;
#104525=EDGE_CURVE ( 'NONE', #12341, #104358, #40381, .T. ) ;
#104526=EDGE_CURVE ( 'NONE', #106999, #2948, #18784, .T. ) ;
#104527=DIRECTION ( 'NONE',  ( 0.000000000000000000, 0.000000000000000000, 1.000000000000000000 ) ) ;
#104528=AXIS2_PLACEMENT_3D ( 'NONE', #82927, #12228, #80985 ) ;
#104529=EDGE_CURVE ( 'NONE', #44872, #51386, #92600, .T. ) ;
#104530=ORIENTED_EDGE ( 'NONE', *, *, #25147, .F. ) ;
#104531=ORIENTED_EDGE ( 'NONE', *, *, #72897, .F. ) ;
#104532=CIRCLE ( 'NONE', #114982, 0.06509327318403745899 ) ;
#104533=CARTESIAN_POINT ( 'NONE',  ( -14.34999999999998543, 2.500000000000000000, -1.818653347947323695 ) ) ;
#104534=AXIS2_PLACEMENT_3D ( 'NONE', #99635, #20425, #2700 ) ;
#104535=PLANE ( 'NONE',  #22309 ) ;
#104536=EDGE_CURVE ( 'NONE', #24357, #78982, #3005, .T. ) ;
#104537=DIRECTION ( 'NONE',  ( 0.000000000000000000, 0.000000000000000000, -1.000000000000000000 ) ) ;
#104538=ORIENTED_EDGE ( 'NONE', *, *, #11726, .T. ) ;
#104539=ORIENTED_EDGE ( 'NONE', *, *, #45093, .T. ) ;
#104540=ADVANCED_FACE ( 'NONE', ( #86883 ), #18142, .T. ) ;
#104541=CARTESIAN_POINT ( 'NONE',  ( -5.850000000000021849, 2.500000000000000000, -5.802370205355749988 ) ) ;
#104543=ORIENTED_EDGE ( 'NONE', *, *, #68193, .T. ) ;
#104544=CARTESIAN_POINT ( 'NONE',  ( -4.600000000000025402, 2.500000000000000000, -2.385244779468109755E-15 ) ) ;
#104545=EDGE_CURVE ( 'NONE', #79392, #85331, #126030, .T. ) ;
#104546=ADVANCED_FACE ( 'NONE', ( #97992 ), #113523, .T. ) ;
#104547=DIRECTION ( 'NONE',  ( 0.000000000000000000, 0.000000000000000000, 1.000000000000000000 ) ) ;
#104548=EDGE_LOOP ( 'NONE', ( #73421, #62273, #9171, #75575 ) ) ;
#104549=DIRECTION ( 'NONE',  ( 0.000000000000000000, 0.000000000000000000, 1.000000000000000000 ) ) ;
#104550=CARTESIAN_POINT ( 'NONE',  ( 5.399999999999934630, 2.500000000000000000, -0.5928203230275542746 ) ) ;
#104551=AXIS2_PLACEMENT_3D ( 'NONE', #120420, #60853, #109960 ) ;
#104552=DIRECTION ( 'NONE',  ( 0.000000000000000000, 1.000000000000000000, 0.000000000000000000 ) ) ;
#104553=CARTESIAN_POINT ( 'NONE',  ( 1.049999999999953637, 12.50000000000000000, -1.818653347947326138 ) ) ;
#104554=EDGE_CURVE ( 'NONE', #48799, #105604, #57085, .T. ) ;
#104555=ORIENTED_EDGE ( 'NONE', *, *, #106869, .T. ) ;
#104556=DIRECTION ( 'NONE',  ( -0.000000000000000000, -1.000000000000000000, -0.000000000000000000 ) ) ;
#104557=FACE_OUTER_BOUND ( 'NONE', #51737, .T. ) ;
#104558=ORIENTED_EDGE ( 'NONE', *, *, #10262, .F. ) ;
#104559=ORIENTED_EDGE ( 'NONE', *, *, #65676, .F. ) ;
#104560=LINE ( 'NONE', #126131, #4461 ) ;
#104561=DIRECTION ( 'NONE',  ( 0.000000000000000000, 1.000000000000000000, 0.000000000000000000 ) ) ;
#104563=DIRECTION ( 'NONE',  ( 0.000000000000000000, 0.000000000000000000, 1.000000000000000000 ) ) ;
#104564=CARTESIAN_POINT ( 'NONE',  ( -0.4500000000000402012, 2.500000000000000000, 6.395190528383296602 ) ) ;
#104565=DIRECTION ( 'NONE',  ( 0.000000000000000000, 0.000000000000000000, -1.000000000000000000 ) ) ;
#104566=DIRECTION ( 'NONE',  ( 0.000000000000000000, -0.9999939076577903929, 0.003490651415223739937 ) ) ;
#104567=FACE_OUTER_BOUND ( 'NONE', #116001, .T. ) ;
#104568=CARTESIAN_POINT ( 'NONE',  ( -5.450000000000023270, 2.500000000000000000, -6.395190528383301931 ) ) ;
#104569=CONICAL_SURFACE ( 'NONE', #20943, 0.09999999999999982514, 0.003490658503988666988 ) ;
#104570=CIRCLE ( 'NONE', #6338, 0.06509327318403745899 ) ;
#104571=DIRECTION ( 'NONE',  ( 0.000000000000000000, -0.9999939076577903929, 0.003490651415223739937 ) ) ;
#104572=EDGE_LOOP ( 'NONE', ( #65576, #121503 ) ) ;
#104573=ORIENTED_EDGE ( 'NONE', *, *, #74412, .F. ) ;
#104574=CIRCLE ( 'NONE', #48147, 0.06509327318403745899 ) ;
#104575=VERTEX_POINT ( 'NONE', #40385 ) ;
#104576=VERTEX_POINT ( 'NONE', #1719 ) ;
#104577=DIRECTION ( 'NONE',  ( 0.000000000000000000, -0.000000000000000000, 1.000000000000000000 ) ) ;
#104578=CARTESIAN_POINT ( 'NONE',  ( 12.89999999999989733, 12.50000000000000000, -2.385244779468109755E-15 ) ) ;
#104579=DIRECTION ( 'NONE',  ( -4.274815082592931898E-19, -0.9999939076577903929, -0.003490651415223739937 ) ) ;
#104580=ORIENTED_EDGE ( 'NONE', *, *, #107985, .T. ) ;
#104581=DIRECTION ( 'NONE',  ( -0.000000000000000000, -1.000000000000000000, -0.000000000000000000 ) ) ;
#104582=ADVANCED_FACE ( 'NONE', ( #1084 ), #6884, .T. ) ;
#104583=EDGE_CURVE ( 'NONE', #57277, #116085, #61307, .T. ) ;
#104584=CARTESIAN_POINT ( 'NONE',  ( 4.349999999999939249, 2.500000000000000000, 2.511473670974873507 ) ) ;
#104585=DIRECTION ( 'NONE',  ( 0.000000000000000000, 1.000000000000000000, 0.000000000000000000 ) ) ;
#104586=ORIENTED_EDGE ( 'NONE', *, *, #17666, .F. ) ;
#104587=CARTESIAN_POINT ( 'NONE',  ( -4.200000000000029488, 12.50000000000000000, -4.330127018922201643 ) ) ;
#104588=ORIENTED_EDGE ( 'NONE', *, *, #39669, .F. ) ;
#104589=ADVANCED_FACE ( 'NONE', ( #424 ), #30208, .T. ) ;
#104590=ORIENTED_EDGE ( 'NONE', *, *, #118875, .F. ) ;
#104591=ORIENTED_EDGE ( 'NONE', *, *, #6387, .T. ) ;
#104592=EDGE_LOOP ( 'NONE', ( #45788, #96716, #57972, #76385 ) ) ;
#104593=LINE ( 'NONE', #84953, #53085 ) ;
#104594=DIRECTION ( 'NONE',  ( 0.000000000000000000, -0.9999939076577903929, 0.003490651415223739937 ) ) ;
#104595=CARTESIAN_POINT ( 'NONE',  ( 3.749999999999944045, 12.50000000000000000, -7.188010851410854052 ) ) ;
#104596=FACE_OUTER_BOUND ( 'NONE', #99706, .T. ) ;
#104597=VECTOR ( 'NONE', #84415, 1000.000000000000000 ) ;
#104598=VERTEX_POINT ( 'NONE', #80306 ) ;
#104599=VECTOR ( 'NONE', #70577, 1000.000000000000000 ) ;
#104600=CARTESIAN_POINT ( 'NONE',  ( 9.399999999999915090, 2.500000000000000000, 4.676537180435972552 ) ) ;
#104601=VERTEX_POINT ( 'NONE', #80948 ) ;
#104602=CARTESIAN_POINT ( 'NONE',  ( 8.749999999999918288, 2.500000000000000000, 7.088010851410848190 ) ) ;
#104603=DIRECTION ( 'NONE',  ( 0.000000000000000000, 0.000000000000000000, 1.000000000000000000 ) ) ;
#104604=DIRECTION ( 'NONE',  ( 0.000000000000000000, 0.000000000000000000, 1.000000000000000000 ) ) ;
#104605=LINE ( 'NONE', #74512, #84038 ) ;
#104606=AXIS2_PLACEMENT_3D ( 'NONE', #94621, #53432, #74998 ) ;
#104607=EDGE_LOOP ( 'NONE', ( #104973, #46406 ) ) ;
#104608=VERTEX_POINT ( 'NONE', #12814 ) ;
#104609=EDGE_LOOP ( 'NONE', ( #80374, #111713 ) ) ;
#104610=LINE ( 'NONE', #14912, #44005 ) ;
#104611=DIRECTION ( 'NONE',  ( -0.000000000000000000, 1.000000000000000000, -0.000000000000000000 ) ) ;
#104612=PLANE ( 'NONE',  #16859 ) ;
#104613=FACE_BOUND ( 'NONE', #125175, .T. ) ;
#104614=CARTESIAN_POINT ( 'NONE',  ( 6.649999999999930189, 12.50000000000000000, 5.802370205355744659 ) ) ;
#104615=CARTESIAN_POINT ( 'NONE',  ( 3.549999999999943867, 12.50000000000000000, -1.818653347947326138 ) ) ;
#104616=PLANE ( 'NONE',  #29108 ) ;
#104617=AXIS2_PLACEMENT_3D ( 'NONE', #85750, #15049, #17654 ) ;
#104618=EDGE_CURVE ( 'NONE', #71554, #126826, #52895, .T. ) ;
#104619=CIRCLE ( 'NONE', #100424, 0.06509327318403745899 ) ;
#104621=DIRECTION ( 'NONE',  ( 0.000000000000000000, 0.000000000000000000, 1.000000000000000000 ) ) ;
#104622=DIRECTION ( 'NONE',  ( -4.274815082592931898E-19, -0.9999939076577903929, -0.003490651415223739937 ) ) ;
#104623=ORIENTED_EDGE ( 'NONE', *, *, #40193, .F. ) ;
#104624=AXIS2_PLACEMENT_3D ( 'NONE', #98811, #49097, #119107 ) ;
#104625=FACE_OUTER_BOUND ( 'NONE', #97351, .T. ) ;
#104626=ORIENTED_EDGE ( 'NONE', *, *, #7892, .T. ) ;
#104627=CONICAL_SURFACE ( 'NONE', #79603, 0.1000000000000002554, 0.003490658503988666988 ) ;
#104628=ORIENTED_EDGE ( 'NONE', *, *, #118583, .T. ) ;
#104629=ORIENTED_EDGE ( 'NONE', *, *, #63600, .F. ) ;
#104630=ORIENTED_EDGE ( 'NONE', *, *, #15107, .T. ) ;
#104631=EDGE_CURVE ( 'NONE', #124173, #108711, #29907, .T. ) ;
#104632=DIRECTION ( 'NONE',  ( 0.000000000000000000, 0.000000000000000000, 1.000000000000000000 ) ) ;
#104633=FACE_BOUND ( 'NONE', #52558, .T. ) ;
#104634=CARTESIAN_POINT ( 'NONE',  ( 0.8499999999999536815, 2.500000000000000000, 6.595190528383296780 ) ) ;
#104635=EDGE_LOOP ( 'NONE', ( #33208, #61388, #33348, #72204 ) ) ;
#104636=CARTESIAN_POINT ( 'NONE',  ( 23.99354682432708330, 2.839181451644113618, 2.508508607402079260 ) ) ;
#104637=EDGE_CURVE ( 'NONE', #57040, #92171, #128416, .T. ) ;
#104638=CARTESIAN_POINT ( 'NONE',  ( 8.349999999999919709, 2.500000000000000000, -2.857883832488653741 ) ) ;
#104639=ORIENTED_EDGE ( 'NONE', *, *, #114426, .T. ) ;
#104640=DIRECTION ( 'NONE',  ( 0.000000000000000000, 0.000000000000000000, 1.000000000000000000 ) ) ;
#104641=PLANE ( 'NONE',  #55366 ) ;
#104642=ORIENTED_EDGE ( 'NONE', *, *, #59953, .F. ) ;
#104643=AXIS2_PLACEMENT_3D ( 'NONE', #23762, #85871, #113420 ) ;
#104644=FACE_OUTER_BOUND ( 'NONE', #116273, .T. ) ;
#104645=CIRCLE ( 'NONE', #33656, 0.06509327318403745899 ) ;
#104646=CARTESIAN_POINT ( 'NONE',  ( -10.85000000000000142, 2.500000000000000000, -2.065063509461098068 ) ) ;
#104647=ORIENTED_EDGE ( 'NONE', *, *, #55259, .F. ) ;
#104648=DIRECTION ( 'NONE',  ( 0.000000000000000000, 0.000000000000000000, -1.000000000000000000 ) ) ;
#104651=DIRECTION ( 'NONE',  ( 0.000000000000000000, 1.000000000000000000, 0.000000000000000000 ) ) ;
#104652=VERTEX_POINT ( 'NONE', #101871 ) ;
#104653=AXIS2_PLACEMENT_3D ( 'NONE', #70409, #52067, #31777 ) ;
#104654=ORIENTED_EDGE ( 'NONE', *, *, #46969, .T. ) ;
#104655=DIRECTION ( 'NONE',  ( 0.000000000000000000, 0.000000000000000000, 1.000000000000000000 ) ) ;
#104656=VERTEX_POINT ( 'NONE', #31212 ) ;
#104657=FACE_OUTER_BOUND ( 'NONE', #49400, .T. ) ;
#104658=CARTESIAN_POINT ( 'NONE',  ( 15.59999999999988951, 12.50000000000000000, -0.4115034346978157509 ) ) ;
#104659=EDGE_CURVE ( 'NONE', #3256, #115958, #71970, .T. ) ;
#104660=ORIENTED_EDGE ( 'NONE', *, *, #120394, .T. ) ;
#104661=FACE_OUTER_BOUND ( 'NONE', #79178, .T. ) ;
#104663=CARTESIAN_POINT ( 'NONE',  ( 6.249999999999930722, 12.50000000000000000, 7.188010851410848723 ) ) ;
#104664=DIRECTION ( 'NONE',  ( 0.000000000000000000, 0.000000000000000000, -1.000000000000000000 ) ) ;
#104665=ADVANCED_FACE ( 'NONE', ( #2348 ), #48986, .T. ) ;
#104666=CARTESIAN_POINT ( 'NONE',  ( -0.4000000000000396572, 2.500000000000000000, 4.430127018922196847 ) ) ;
#104667=ADVANCED_FACE ( 'NONE', ( #99941 ), #42745, .T. ) ;
#104668=ORIENTED_EDGE ( 'NONE', *, *, #77795, .T. ) ;
#104669=VERTEX_POINT ( 'NONE', #50207 ) ;
#104670=PLANE ( 'NONE',  #129007 ) ;
#104671=DIRECTION ( 'NONE',  ( 0.000000000000000000, -0.9999939076577903929, 0.003490651415223739937 ) ) ;
#104672=ADVANCED_FACE ( 'NONE', ( #41037 ), #111014, .T. ) ;
#104673=CARTESIAN_POINT ( 'NONE',  ( -7.500000000000015099, 2.500000000000000000, -4.922947341949753586 ) ) ;
#104674=ORIENTED_EDGE ( 'NONE', *, *, #103558, .F. ) ;
#104675=ORIENTED_EDGE ( 'NONE', *, *, #67888, .F. ) ;
#104676=EDGE_CURVE ( 'NONE', #74488, #70177, #110390, .T. ) ;
#104677=VERTEX_POINT ( 'NONE', #70473 ) ;
#104678=ADVANCED_FACE ( 'NONE', ( #20734 ), #31845, .T. ) ;
#104679=FACE_OUTER_BOUND ( 'NONE', #76025, .T. ) ;
#104680=CIRCLE ( 'NONE', #27311, 0.06509327318403741736 ) ;
#104681=CARTESIAN_POINT ( 'NONE',  ( -11.64999999999999680, 12.50000000000000000, 2.857883832488649301 ) ) ;
#104682=CONICAL_SURFACE ( 'NONE', #106829, 0.09999999999999982514, 0.003490658503988666988 ) ;
#104683=CARTESIAN_POINT ( 'NONE',  ( -4.350000000000023626, 12.50000000000000000, 1.883746621131358934 ) ) ;
#104684=EDGE_CURVE ( 'NONE', #101605, #77155, #36273, .T. ) ;
#104685=CARTESIAN_POINT ( 'NONE',  ( -2.300000000000033573, 2.500000000000000000, 4.776537180435972196 ) ) ;
#104686=DIRECTION ( 'NONE',  ( 0.000000000000000000, 0.000000000000000000, 1.000000000000000000 ) ) ;
#104687=PLANE ( 'NONE',  #84140 ) ;
#104688=CARTESIAN_POINT ( 'NONE',  ( 6.049999999999935874, 2.500000000000000000, -6.841600689897077814 ) ) ;
#104689=FACE_OUTER_BOUND ( 'NONE', #114953, .T. ) ;
#104690=DIRECTION ( 'NONE',  ( 0.000000000000000000, 0.000000000000000000, 1.000000000000000000 ) ) ;
#104691=AXIS2_PLACEMENT_3D ( 'NONE', #96071, #6370, #27314 ) ;
#104692=EDGE_CURVE ( 'NONE', #19953, #105928, #78019, .T. ) ;
#104693=CONICAL_SURFACE ( 'NONE', #235, 0.09999999999999982514, 0.003490658503988666988 ) ;
#104694=EDGE_LOOP ( 'NONE', ( #16808, #71632 ) ) ;
#104695=DIRECTION ( 'NONE',  ( -4.274815082592931898E-19, -0.9999939076577903929, -0.003490651415223739937 ) ) ;
#104696=ORIENTED_EDGE ( 'NONE', *, *, #59789, .T. ) ;
#104697=VERTEX_POINT ( 'NONE', #62600 ) ;
#104698=CARTESIAN_POINT ( 'NONE',  ( 7.299999999999926104, 2.500000000000000000, 4.676537180435972552 ) ) ;
#104699=DIRECTION ( 'NONE',  ( 0.000000000000000000, 1.000000000000000000, 0.000000000000000000 ) ) ;
#104700=CARTESIAN_POINT ( 'NONE',  ( -13.74999999999998934, 2.500000000000000000, -1.372243186433547812 ) ) ;
#104701=CIRCLE ( 'NONE', #48290, 0.06509327318403743123 ) ;
#104702=DIRECTION ( 'NONE',  ( 0.000000000000000000, -0.000000000000000000, 1.000000000000000000 ) ) ;
#104703=VECTOR ( 'NONE', #93359, 1000.000000000000000 ) ;
#104705=CARTESIAN_POINT ( 'NONE',  ( 12.89999999999989910, 2.500000000000000000, -0.6928203230275542523 ) ) ;
#104706=FACE_OUTER_BOUND ( 'NONE', #19028, .T. ) ;
#104707=DIRECTION ( 'NONE',  ( -0.000000000000000000, -1.000000000000000000, -0.000000000000000000 ) ) ;
#104708=ORIENTED_EDGE ( 'NONE', *, *, #44863, .F. ) ;
#104709=DIRECTION ( 'NONE',  ( 0.000000000000000000, 0.000000000000000000, -1.000000000000000000 ) ) ;
#104710=CONICAL_SURFACE ( 'NONE', #94257, 0.09999999999999982514, 0.003490658503988666988 ) ;
#104711=CARTESIAN_POINT ( 'NONE',  ( -0.8500000000000395017, 2.500000000000000000, 6.595190528383296780 ) ) ;
#104713=ORIENTED_EDGE ( 'NONE', *, *, #49032, .F. ) ;
#104714=CIRCLE ( 'NONE', #79684, 0.06509327318403745899 ) ;
#104715=EDGE_LOOP ( 'NONE', ( #75472, #123087 ) ) ;
#104716=VERTEX_POINT ( 'NONE', #89469 ) ;
#104717=PLANE ( 'NONE',  #21158 ) ;
#104718=DIRECTION ( 'NONE',  ( 0.000000000000000000, 0.000000000000000000, -1.000000000000000000 ) ) ;
#104720=ADVANCED_FACE ( 'NONE', ( #129428 ), #39752, .T. ) ;
#104721=FACE_OUTER_BOUND ( 'NONE', #99297, .T. ) ;
#104722=CARTESIAN_POINT ( 'NONE',  ( 17.50000000000000000, 2.500000000000000000, 4.000000000000000888 ) ) ;
#104723=ORIENTED_EDGE ( 'NONE', *, *, #57247, .T. ) ;
#104724=DIRECTION ( 'NONE',  ( -0.000000000000000000, 1.000000000000000000, -0.000000000000000000 ) ) ;
#104725=DIRECTION ( 'NONE',  ( 0.000000000000000000, 0.000000000000000000, 1.000000000000000000 ) ) ;
#104726=DIRECTION ( 'NONE',  ( 0.000000000000000000, 1.000000000000000000, 0.000000000000000000 ) ) ;
#104727=EDGE_CURVE ( 'NONE', #94262, #58821, #23746, .T. ) ;
#104728=ORIENTED_EDGE ( 'NONE', *, *, #108417, .F. ) ;
#104729=ORIENTED_EDGE ( 'NONE', *, *, #97582, .F. ) ;
#104730=ORIENTED_EDGE ( 'NONE', *, *, #38854, .T. ) ;
#104731=CONICAL_SURFACE ( 'NONE', #40015, 0.1000000000000002554, 0.003490658503988666988 ) ;
#104732=CARTESIAN_POINT ( 'NONE',  ( 8.549999999999924327, 12.50000000000000000, 1.818653347947321475 ) ) ;
#104733=CONICAL_SURFACE ( 'NONE', #54560, 0.09999999999999982514, 0.003490658503988666988 ) ;
#104734=CARTESIAN_POINT ( 'NONE',  ( -3.749999999999991118, 12.50000000000000000, 2.165063509461097713 ) ) ;
#104736=AXIS2_PLACEMENT_3D ( 'NONE', #74020, #62909, #43286 ) ;
#104737=ORIENTED_EDGE ( 'NONE', *, *, #79570, .F. ) ;
#104738=DIRECTION ( 'NONE',  ( 0.000000000000000000, 1.000000000000000000, 0.000000000000000000 ) ) ;
#104739=DIRECTION ( 'NONE',  ( -0.000000000000000000, 1.000000000000000000, -0.000000000000000000 ) ) ;
#104740=CARTESIAN_POINT ( 'NONE',  ( 9.549999999999918998, 12.50000000000000000, 2.099970236277060032 ) ) ;
#104741=DIRECTION ( 'NONE',  ( 0.000000000000000000, 1.000000000000000000, 0.000000000000000000 ) ) ;
#104742=LINE ( 'NONE', #104125, #89585 ) ;
#104743=ORIENTED_EDGE ( 'NONE', *, *, #88633, .T. ) ;
#104744=DIRECTION ( 'NONE',  ( 0.000000000000000000, 1.000000000000000000, 0.000000000000000000 ) ) ;
#104745=VERTEX_POINT ( 'NONE', #84144 ) ;
#104746=EDGE_LOOP ( 'NONE', ( #35606, #43651 ) ) ;
#104747=DIRECTION ( 'NONE',  ( 0.000000000000000000, 0.000000000000000000, -1.000000000000000000 ) ) ;
#104748=FACE_BOUND ( 'NONE', #124439, .T. ) ;
#104749=DIRECTION ( 'NONE',  ( 0.000000000000000000, 0.000000000000000000, 1.000000000000000000 ) ) ;
#104750=CARTESIAN_POINT ( 'NONE',  ( -4.250072516143177381E-14, 12.50000000000000000, -3.637306695894650055 ) ) ;
#104751=DIRECTION ( 'NONE',  ( 0.000000000000000000, 0.000000000000000000, 1.000000000000000000 ) ) ;
#104752=EDGE_CURVE ( 'NONE', #57522, #26422, #115663, .T. ) ;
#104753=ORIENTED_EDGE ( 'NONE', *, *, #11567, .F. ) ;
#104754=EDGE_LOOP ( 'NONE', ( #65761, #44802, #58976, #115435 ) ) ;
#104755=CARTESIAN_POINT ( 'NONE',  ( -6.650000000000019007, 12.50000000000000000, -5.737276932171712751 ) ) ;
#104756=EDGE_CURVE ( 'NONE', #70003, #55669, #74339, .T. ) ;
#104757=LINE ( 'NONE', #15079, #36305 ) ;
#104758=LINE ( 'NONE', #107359, #50792 ) ;
#104759=LINE ( 'NONE', #46499, #23885 ) ;
#104760=ORIENTED_EDGE ( 'NONE', *, *, #67851, .F. ) ;
#104761=CIRCLE ( 'NONE', #96360, 0.1000000000000000472 ) ;
#104762=EDGE_CURVE ( 'NONE', #80302, #88979, #92688, .T. ) ;
#104763=DIRECTION ( 'NONE',  ( -0.000000000000000000, 1.000000000000000000, -0.000000000000000000 ) ) ;
#104764=AXIS2_PLACEMENT_3D ( 'NONE', #35658, #27125, #65747 ) ;
#104765=DIRECTION ( 'NONE',  ( 0.000000000000000000, 0.000000000000000000, -1.000000000000000000 ) ) ;
#104766=VERTEX_POINT ( 'NONE', #114259 ) ;
#104767=EDGE_CURVE ( 'NONE', #57867, #51861, #82886, .T. ) ;
#104768=CARTESIAN_POINT ( 'NONE',  ( 6.849999999999929479, 12.50000000000000000, -2.511473670974877948 ) ) ;
#104769=EDGE_CURVE ( 'NONE', #56167, #113064, #57179, .T. ) ;
#104770=EDGE_LOOP ( 'NONE', ( #68245, #129179, #108776, #19199 ) ) ;
#104771=FACE_BOUND ( 'NONE', #29254, .T. ) ;
#104772=CONICAL_SURFACE ( 'NONE', #121498, 0.09999999999999982514, 0.003490658503988666988 ) ;
#104773=LINE ( 'NONE', #22389, #57896 ) ;
#104774=AXIS2_PLACEMENT_3D ( 'NONE', #19564, #49689, #110519 ) ;
#104775=VERTEX_POINT ( 'NONE', #33140 ) ;
#104776=CARTESIAN_POINT ( 'NONE',  ( 7.099999999999928590, 2.500000000000000000, -4.922947341949753586 ) ) ;
#104777=DIRECTION ( 'NONE',  ( 0.000000000000000000, -0.9999939076577903929, 0.003490651415223739937 ) ) ;
#104778=EDGE_CURVE ( 'NONE', #8315, #44421, #52981, .T. ) ;
#104779=ORIENTED_EDGE ( 'NONE', *, *, #113099, .F. ) ;
#104780=EDGE_LOOP ( 'NONE', ( #116379, #129293 ) ) ;
#104781=EDGE_CURVE ( 'NONE', #81044, #69509, #71764, .T. ) ;
#104783=AXIS2_PLACEMENT_3D ( 'NONE', #119563, #129430, #88155 ) ;
#104785=DIRECTION ( 'NONE',  ( -0.000000000000000000, 1.000000000000000000, -0.000000000000000000 ) ) ;
#104786=AXIS2_PLACEMENT_3D ( 'NONE', #127341, #126687, #96556 ) ;
#104787=CARTESIAN_POINT ( 'NONE',  ( 5.449999999999934452, 2.500000000000000000, 2.165063509461097713 ) ) ;
#104788=VECTOR ( 'NONE', #22669, 1000.000000000000000 ) ;
#104789=CARTESIAN_POINT ( 'NONE',  ( -3.642919299551294898E-14, 2.500000000000000000, 0.6928203230275518099 ) ) ;
#104790=DIRECTION ( 'NONE',  ( -4.274815082592931898E-19, -0.9999939076577903929, -0.003490651415223739937 ) ) ;
#104791=DIRECTION ( 'NONE',  ( 0.000000000000000000, 0.000000000000000000, 1.000000000000000000 ) ) ;
#104792=AXIS2_PLACEMENT_3D ( 'NONE', #63900, #104461, #74362 ) ;
#104793=EDGE_LOOP ( 'NONE', ( #96210, #74189, #128577, #13719 ) ) ;
#104794=ORIENTED_EDGE ( 'NONE', *, *, #8365, .T. ) ;
#104795=CARTESIAN_POINT ( 'NONE',  ( -3.750000000000027534, 12.50000000000000000, 2.922977105672686982 ) ) ;
#104796=AXIS2_PLACEMENT_3D ( 'NONE', #10608, #110125, #19140 ) ;
#104797=VECTOR ( 'NONE', #125473, 1000.000000000000000 ) ;
#104798=DIRECTION ( 'NONE',  ( 0.000000000000000000, 0.000000000000000000, -1.000000000000000000 ) ) ;
#104799=DIRECTION ( 'NONE',  ( -0.000000000000000000, -1.000000000000000000, -0.000000000000000000 ) ) ;
#104800=DIRECTION ( 'NONE',  ( -0.000000000000000000, 1.000000000000000000, -0.000000000000000000 ) ) ;
#104801=VERTEX_POINT ( 'NONE', #54056 ) ;
#104802=ORIENTED_EDGE ( 'NONE', *, *, #82999, .T. ) ;
#104803=FACE_BOUND ( 'NONE', #63894, .T. ) ;
#104804=ORIENTED_EDGE ( 'NONE', *, *, #45404, .T. ) ;
#104806=DIRECTION ( 'NONE',  ( 0.000000000000000000, 1.000000000000000000, 0.000000000000000000 ) ) ;
#104807=EDGE_LOOP ( 'NONE', ( #95716, #19890, #121291, #67423 ) ) ;
#104808=DIRECTION ( 'NONE',  ( 0.000000000000000000, 1.000000000000000000, 0.000000000000000000 ) ) ;
#104809=CARTESIAN_POINT ( 'NONE',  ( -5.200000000000022382, 2.500000000000000000, 4.576537180435972019 ) ) ;
#104810=ADVANCED_FACE ( 'NONE', ( #83528 ), #67533, .T. ) ;
#104812=DIRECTION ( 'NONE',  ( -0.000000000000000000, 1.000000000000000000, -0.000000000000000000 ) ) ;
#104813=CARTESIAN_POINT ( 'NONE',  ( -8.750000000000007105, 12.50000000000000000, 7.188010851410848723 ) ) ;
#104814=DIRECTION ( 'NONE',  ( 0.000000000000000000, 1.000000000000000000, 0.000000000000000000 ) ) ;
#104816=DIRECTION ( 'NONE',  ( 0.000000000000000000, 0.000000000000000000, -1.000000000000000000 ) ) ;
#104817=PLANE ( 'NONE',  #107892 ) ;
#104818=EDGE_CURVE ( 'NONE', #52810, #91937, #55345, .T. ) ;
#104819=EDGE_LOOP ( 'NONE', ( #21904, #36719 ) ) ;
#104821=VERTEX_POINT ( 'NONE', #23292 ) ;
#104822=DIRECTION ( 'NONE',  ( 0.000000000000000000, 0.000000000000000000, -1.000000000000000000 ) ) ;
#104823=EDGE_LOOP ( 'NONE', ( #21149, #44459 ) ) ;
#104824=AXIS2_PLACEMENT_3D ( 'NONE', #33963, #73882, #32698 ) ;
#104825=CARTESIAN_POINT ( 'NONE',  ( 21.24754738303277435, 0.7337760880902381988, 4.182111650399361835 ) ) ;
#104826=AXIS2_PLACEMENT_3D ( 'NONE', #107136, #67861, #106504 ) ;
#104827=EDGE_CURVE ( 'NONE', #11852, #45708, #42537, .T. ) ;
#104828=AXIS2_PLACEMENT_3D ( 'NONE', #21154, #2809, #80741 ) ;
#104829=VERTEX_POINT ( 'NONE', #45536 ) ;
#104830=VERTEX_POINT ( 'NONE', #93339 ) ;
#104831=ORIENTED_EDGE ( 'NONE', *, *, #80772, .T. ) ;
#104832=ADVANCED_FACE ( 'NONE', ( #125374 ), #25218, .T. ) ;
#104833=FACE_OUTER_BOUND ( 'NONE', #37120, .T. ) ;
#104834=EDGE_CURVE ( 'NONE', #127971, #13889, #75953, .T. ) ;
#104835=AXIS2_PLACEMENT_3D ( 'NONE', #41845, #22208, #12987 ) ;
#104836=CARTESIAN_POINT ( 'NONE',  ( -1.250000000000037970, 2.500000000000000000, 7.088010851410848190 ) ) ;
#104837=CIRCLE ( 'NONE', #33747, 0.06509327318403741736 ) ;
#104839=EDGE_CURVE ( 'NONE', #84139, #4806, #25785, .T. ) ;
#104840=CARTESIAN_POINT ( 'NONE',  ( -5.650000000000019895, 2.500000000000000000, 6.248780366869520542 ) ) ;
#104841=DIRECTION ( 'NONE',  ( -4.274815082592931898E-19, -0.9999939076577903929, -0.003490651415223739937 ) ) ;
#104842=CIRCLE ( 'NONE', #105026, 0.1000000000000000472 ) ;
#104843=DIRECTION ( 'NONE',  ( 0.000000000000000000, -0.000000000000000000, 1.000000000000000000 ) ) ;
#104844=ORIENTED_EDGE ( 'NONE', *, *, #53840, .T. ) ;
#104845=CARTESIAN_POINT ( 'NONE',  ( -9.350000000000006750, 2.500000000000000000, -1.818653347947325916 ) ) ;
#104846=EDGE_CURVE ( 'NONE', #122810, #89858, #113620, .T. ) ;
#104847=AXIS2_PLACEMENT_3D ( 'NONE', #69722, #109651, #67103 ) ;
#104848=ORIENTED_EDGE ( 'NONE', *, *, #128523, .F. ) ;
#104849=EDGE_CURVE ( 'NONE', #66518, #13897, #13253, .T. ) ;
#104850=EDGE_LOOP ( 'NONE', ( #72147, #96601, #115675, #26039 ) ) ;
#104851=ORIENTED_EDGE ( 'NONE', *, *, #31174, .F. ) ;
#104852=CARTESIAN_POINT ( 'NONE',  ( -1.700000000000034817, 12.50000000000000000, -2.385244779468109755E-15 ) ) ;
#104853=VERTEX_POINT ( 'NONE', #54672 ) ;
#104854=VERTEX_POINT ( 'NONE', #105070 ) ;
#104855=EDGE_LOOP ( 'NONE', ( #15833, #55528 ) ) ;
#104856=CARTESIAN_POINT ( 'NONE',  ( 7.699999999999923794, 12.50000000000000000, 4.611443907251934426 ) ) ;
#104857=DIRECTION ( 'NONE',  ( 0.000000000000000000, -0.000000000000000000, 1.000000000000000000 ) ) ;
#104858=FACE_OUTER_BOUND ( 'NONE', #27474, .T. ) ;
#104859=CARTESIAN_POINT ( 'NONE',  ( 2.899999999999945732, 2.500000000000000000, -4.330127018922201643 ) ) ;
#104860=CARTESIAN_POINT ( 'NONE',  ( 12.93920187831608892, 1.500000000000000222, 10.00000000000000000 ) ) ;
#104861=EDGE_LOOP ( 'NONE', ( #59171, #92034, #121907, #63175 ) ) ;
#104862=FACE_OUTER_BOUND ( 'NONE', #2473, .T. ) ;
#104863=CONICAL_SURFACE ( 'NONE', #17007, 0.1000000000000002554, 0.003490658503988666988 ) ;
#104864=AXIS2_PLACEMENT_3D ( 'NONE', #119215, #69454, #108740 ) ;
#104865=ORIENTED_EDGE ( 'NONE', *, *, #39432, .F. ) ;
#104866=DIRECTION ( 'NONE',  ( 0.000000000000000000, 1.000000000000000000, 0.000000000000000000 ) ) ;
#104868=FACE_OUTER_BOUND ( 'NONE', #38899, .T. ) ;
#104869=EDGE_LOOP ( 'NONE', ( #64780, #92505 ) ) ;
#104870=ORIENTED_EDGE ( 'NONE', *, *, #50513, .T. ) ;
#104871=CIRCLE ( 'NONE', #19090, 0.09999999999999982514 ) ;
#104872=LINE ( 'NONE', #83948, #109634 ) ;
#104873=CARTESIAN_POINT ( 'NONE',  ( 0.3999999999999559464, 2.500000000000000000, -4.230127018922201998 ) ) ;
#104874=CIRCLE ( 'NONE', #113288, 0.1000000000000002554 ) ;
#104876=CARTESIAN_POINT ( 'NONE',  ( 5.599999999999933031, 12.50000000000000000, -0.2813168883297409439 ) ) ;
#104877=DIRECTION ( 'NONE',  ( -0.000000000000000000, 1.000000000000000000, -0.000000000000000000 ) ) ;
#104878=ORIENTED_EDGE ( 'NONE', *, *, #105832, .T. ) ;
#104879=DIRECTION ( 'NONE',  ( 0.000000000000000000, 0.000000000000000000, -1.000000000000000000 ) ) ;
#104880=DIRECTION ( 'NONE',  ( -0.000000000000000000, -1.000000000000000000, -0.000000000000000000 ) ) ;
#104883=DIRECTION ( 'NONE',  ( 0.000000000000000000, 1.000000000000000000, 0.000000000000000000 ) ) ;
#104884=AXIS2_PLACEMENT_3D ( 'NONE', #109614, #8169, #67067 ) ;
#104885=CIRCLE ( 'NONE', #125815, 0.06509327318403745899 ) ;
#104886=CARTESIAN_POINT ( 'NONE',  ( 5.449999999999934452, 12.50000000000000000, 2.099970236277060032 ) ) ;
#104887=ADVANCED_FACE ( 'NONE', ( #4930 ), #46721, .T. ) ;
#104888=ORIENTED_EDGE ( 'NONE', *, *, #26912, .F. ) ;
#104889=AXIS2_PLACEMENT_3D ( 'NONE', #110748, #89824, #87875 ) ;
#104890=CIRCLE ( 'NONE', #14989, 0.09999999999999982514 ) ;
#104891=VECTOR ( 'NONE', #8230, 1000.000000000000000 ) ;
#104892=ORIENTED_EDGE ( 'NONE', *, *, #6304, .F. ) ;
#104893=CIRCLE ( 'NONE', #77701, 0.06509327318403745899 ) ;
#104894=ORIENTED_EDGE ( 'NONE', *, *, #71394, .F. ) ;
#104895=DIRECTION ( 'NONE',  ( 0.000000000000000000, 0.000000000000000000, -1.000000000000000000 ) ) ;
#104896=CARTESIAN_POINT ( 'NONE',  ( -9.999999999999969802, 2.500000000000000000, 4.230127018922196669 ) ) ;
#104897=CIRCLE ( 'NONE', #46415, 0.06509327318403745899 ) ;
#104899=LINE ( 'NONE', #53250, #9256 ) ;
#104900=CARTESIAN_POINT ( 'NONE',  ( 3.949999999999942446, 2.500000000000000000, -2.611473670974877592 ) ) ;
#104901=LINE ( 'NONE', #114098, #108767 ) ;
#104902=LINE ( 'NONE', #85276, #12023 ) ;
#104903=ORIENTED_EDGE ( 'NONE', *, *, #45504, .T. ) ;
#104904=DIRECTION ( 'NONE',  ( 0.000000000000000000, 0.000000000000000000, -1.000000000000000000 ) ) ;
#104906=ORIENTED_EDGE ( 'NONE', *, *, #48516, .T. ) ;
#104907=CARTESIAN_POINT ( 'NONE',  ( -11.64999999999999858, 2.500000000000000000, -5.902370205355746968 ) ) ;
#104908=VERTEX_POINT ( 'NONE', #96531 ) ;
#104909=FACE_OUTER_BOUND ( 'NONE', #20881, .T. ) ;
#104910=CIRCLE ( 'NONE', #121651, 0.06509327318403745899 ) ;
#104911=CIRCLE ( 'NONE', #115367, 0.06509327318403745899 ) ;
#104912=AXIS2_PLACEMENT_3D ( 'NONE', #41951, #81843, #121771 ) ;
#104913=ORIENTED_EDGE ( 'NONE', *, *, #35826, .T. ) ;
#104914=CARTESIAN_POINT ( 'NONE',  ( -14.14999999999998792, 2.500000000000000000, -1.572243186433547990 ) ) ;
#104915=CARTESIAN_POINT ( 'NONE',  ( -9.600000000000008527, 2.500000000000000000, -5.022947341949749678 ) ) ;
#104916=DIRECTION ( 'NONE',  ( 0.000000000000000000, 1.000000000000000000, 0.000000000000000000 ) ) ;
#104917=ORIENTED_EDGE ( 'NONE', *, *, #65780, .F. ) ;
#104918=EDGE_CURVE ( 'NONE', #27344, #22140, #19525, .T. ) ;
#104919=CONICAL_SURFACE ( 'NONE', #121658, 0.09999999999999982514, 0.003490658503988666988 ) ;
#104920=CARTESIAN_POINT ( 'NONE',  ( -9.150000000000009237, 2.500000000000000000, -2.065063509461102065 ) ) ;
#104921=VECTOR ( 'NONE', #16333, 1000.000000000000000 ) ;
#104922=AXIS2_PLACEMENT_3D ( 'NONE', #7281, #96307, #47235 ) ;
#104923=CARTESIAN_POINT ( 'NONE',  ( 6.249999999999930722, 2.500000000000000000, -1.472243186433550122 ) ) ;
#104924=AXIS2_PLACEMENT_3D ( 'NONE', #57190, #18550, #7433 ) ;
#104925=EDGE_CURVE ( 'NONE', #62359, #100751, #73904, .T. ) ;
#104926=ADVANCED_FACE ( 'NONE', ( #97202 ), #17455, .T. ) ;
#104927=ORIENTED_EDGE ( 'NONE', *, *, #26123, .T. ) ;
#104928=AXIS2_PLACEMENT_3D ( 'NONE', #75111, #124209, #65270 ) ;
#104929=DIRECTION ( 'NONE',  ( -0.000000000000000000, 1.000000000000000000, -0.000000000000000000 ) ) ;
#104930=ORIENTED_EDGE ( 'NONE', *, *, #72734, .T. ) ;
#104931=ORIENTED_EDGE ( 'NONE', *, *, #9401, .F. ) ;
#104932=DIRECTION ( 'NONE',  ( 0.000000000000000000, 1.000000000000000000, 0.000000000000000000 ) ) ;
#104933=DIRECTION ( 'NONE',  ( 0.000000000000000000, 0.000000000000000000, -1.000000000000000000 ) ) ;
#104935=ADVANCED_FACE ( 'NONE', ( #106372 ), #113615, .T. ) ;
#104936=ORIENTED_EDGE ( 'NONE', *, *, #3292, .F. ) ;
#104937=EDGE_CURVE ( 'NONE', #30053, #116514, #40484, .T. ) ;
#104938=CARTESIAN_POINT ( 'NONE',  ( 5.199999999999931788, 12.50000000000000000, 4.611443907251934426 ) ) ;
#104939=DIRECTION ( 'NONE',  ( -0.000000000000000000, 1.000000000000000000, -0.000000000000000000 ) ) ;
#104940=ORIENTED_EDGE ( 'NONE', *, *, #12351, .T. ) ;
#104941=LINE ( 'NONE', #36878, #105314 ) ;
#104942=DIRECTION ( 'NONE',  ( 0.000000000000000000, 1.000000000000000000, 0.000000000000000000 ) ) ;
#104943=FACE_OUTER_BOUND ( 'NONE', #102841, .T. ) ;
#104944=DIRECTION ( 'NONE',  ( 0.000000000000000000, 1.000000000000000000, 0.000000000000000000 ) ) ;
#104945=LINE ( 'NONE', #106257, #47234 ) ;
#104946=DIRECTION ( 'NONE',  ( 0.000000000000000000, 0.000000000000000000, -1.000000000000000000 ) ) ;
#104947=CIRCLE ( 'NONE', #397, 0.1000000000000002554 ) ;
#104948=ORIENTED_EDGE ( 'NONE', *, *, #68957, .F. ) ;
#104949=VERTEX_POINT ( 'NONE', #48108 ) ;
#104950=ORIENTED_EDGE ( 'NONE', *, *, #117121, .T. ) ;
#104951=ORIENTED_EDGE ( 'NONE', *, *, #20603, .F. ) ;
#104952=CARTESIAN_POINT ( 'NONE',  ( -0.6000000000000388356, 2.500000000000000000, 4.676537180435972552 ) ) ;
#104953=LINE ( 'NONE', #114786, #54045 ) ;
#104954=DIRECTION ( 'NONE',  ( 0.000000000000000000, 1.000000000000000000, 0.000000000000000000 ) ) ;
#104955=EDGE_LOOP ( 'NONE', ( #89026, #108223 ) ) ;
#104956=FACE_BOUND ( 'NONE', #116496, .T. ) ;
#104957=VECTOR ( 'NONE', #128126, 1000.000000000000000 ) ;
#104958=CARTESIAN_POINT ( 'NONE',  ( -11.24999999999996447, 2.500000000000000000, -6.495190528383298911 ) ) ;
#104959=CARTESIAN_POINT ( 'NONE',  ( -1.450000000000036371, 12.50000000000000000, 2.576566944158910744 ) ) ;
#104960=CIRCLE ( 'NONE', #117563, 0.09999999999999982514 ) ;
#104961=AXIS2_PLACEMENT_3D ( 'NONE', #15195, #76723, #7320 ) ;
#104962=CARTESIAN_POINT ( 'NONE',  ( 6.049999999999934097, 12.50000000000000000, -2.511473670974877948 ) ) ;
#104963=FACE_OUTER_BOUND ( 'NONE', #124076, .T. ) ;
#104964=CARTESIAN_POINT ( 'NONE',  ( 8.949999999999917577, 12.50000000000000000, 6.213873640053558134 ) ) ;
#104965=CARTESIAN_POINT ( 'NONE',  ( 2.949999999999945111, 2.500000000000000000, 2.065063509461097624 ) ) ;
#104966=CARTESIAN_POINT ( 'NONE',  ( 4.399999999999939071, 2.500000000000000000, 0.3464101615137736845 ) ) ;
#104967=CARTESIAN_POINT ( 'NONE',  ( 9.199999999999919353, 12.50000000000000000, -0.06509327318403970719 ) ) ;
#104969=DIRECTION ( 'NONE',  ( 0.000000000000000000, 0.000000000000000000, 1.000000000000000000 ) ) ;
#104970=VECTOR ( 'NONE', #85766, 1000.000000000000000 ) ;
#104971=CARTESIAN_POINT ( 'NONE',  ( 2.499999999999947153, 2.500000000000000000, 0.5928203230275495006 ) ) ;
#104972=CIRCLE ( 'NONE', #79949, 0.09999999999999982514 ) ;
#104973=ORIENTED_EDGE ( 'NONE', *, *, #104659, .T. ) ;
#104974=EDGE_LOOP ( 'NONE', ( #89454, #123507 ) ) ;
#104975=ORIENTED_EDGE ( 'NONE', *, *, #33309, .T. ) ;
#104976=EDGE_LOOP ( 'NONE', ( #81498, #76069, #61452, #36322 ) ) ;
#104978=AXIS2_PLACEMENT_3D ( 'NONE', #92437, #61043, #3416 ) ;
#104979=CARTESIAN_POINT ( 'NONE',  ( -10.40000000000000391, 2.500000000000000000, -3.737306695894645259 ) ) ;
#104980=ORIENTED_EDGE ( 'NONE', *, *, #129554, .F. ) ;
#104981=EDGE_CURVE ( 'NONE', #7558, #10391, #18633, .T. ) ;
#104982=CARTESIAN_POINT ( 'NONE',  ( -14.34999999999998543, 2.500000000000000000, -1.818653347947323695 ) ) ;
#104983=ADVANCED_FACE ( 'NONE', ( #78872 ), #55028, .T. ) ;
#104984=ORIENTED_EDGE ( 'NONE', *, *, #112535, .F. ) ;
#104985=EDGE_LOOP ( 'NONE', ( #102964, #90694, #6081, #123795 ) ) ;
#104986=AXIS2_PLACEMENT_3D ( 'NONE', #87719, #13981, #106713 ) ;
#104987=EDGE_CURVE ( 'NONE', #90431, #76513, #29126, .T. ) ;
#104988=CARTESIAN_POINT ( 'NONE',  ( 5.399999999999934630, 12.50000000000000000, 0.7579135962115869374 ) ) ;
#104989=AXIS2_PLACEMENT_3D ( 'NONE', #94193, #15617, #4490 ) ;
#104990=CARTESIAN_POINT ( 'NONE',  ( 6.598553918451516509, -2.500000000000000888, 8.770211965177990621 ) ) ;
#104991=DIRECTION ( 'NONE',  ( 0.000000000000000000, 0.000000000000000000, -1.000000000000000000 ) ) ;
#104992=DIRECTION ( 'NONE',  ( -0.000000000000000000, -1.000000000000000000, -0.000000000000000000 ) ) ;
#104993=EDGE_CURVE ( 'NONE', #26812, #50137, #88474, .T. ) ;
#104994=CARTESIAN_POINT ( 'NONE',  ( -11.44999999999999751, 12.50000000000000000, 6.841600689897072485 ) ) ;
#104995=EDGE_CURVE ( 'NONE', #88412, #46827, #17989, .T. ) ;
#104996=ORIENTED_EDGE ( 'NONE', *, *, #4625, .T. ) ;
#104997=EDGE_CURVE ( 'NONE', #110014, #76885, #48787, .T. ) ;
#104999=EDGE_LOOP ( 'NONE', ( #15118, #79341 ) ) ;
#105000=EDGE_CURVE ( 'NONE', #23310, #119345, #124074, .T. ) ;
#105001=ORIENTED_EDGE ( 'NONE', *, *, #38027, .F. ) ;
#105002=CARTESIAN_POINT ( 'NONE',  ( -14.39999999999998614, 2.500000000000000000, -0.3464101615137760715 ) ) ;
#105003=ORIENTED_EDGE ( 'NONE', *, *, #102164, .T. ) ;
#105004=CARTESIAN_POINT ( 'NONE',  ( -14.79999999999998295, 12.50000000000000000, -0.3464101615137760715 ) ) ;
#105005=EDGE_LOOP ( 'NONE', ( #82314, #20496 ) ) ;
#105006=ORIENTED_EDGE ( 'NONE', *, *, #70170, .F. ) ;
#105007=ADVANCED_FACE ( 'NONE', ( #87998 ), #86065, .T. ) ;
#105008=CARTESIAN_POINT ( 'NONE',  ( 6.649999999999929301, 2.500000000000000000, 6.395190528383296602 ) ) ;
#105009=CARTESIAN_POINT ( 'NONE',  ( 1.449999999999951772, 12.50000000000000000, -6.213873640053564351 ) ) ;
#105010=CARTESIAN_POINT ( 'NONE',  ( -1.250000000000035749, 2.500000000000000000, -7.188010851410854052 ) ) ;
#105011=CONICAL_SURFACE ( 'NONE', #59062, 0.1000000000000000472, 0.003490658503988666988 ) ;
#105012=DIRECTION ( 'NONE',  ( -0.000000000000000000, 1.000000000000000000, -0.000000000000000000 ) ) ;
#105013=VECTOR ( 'NONE', #28214, 1000.000000000000000 ) ;
#105014=AXIS2_PLACEMENT_3D ( 'NONE', #95551, #97477, #87008 ) ;
#105015=DIRECTION ( 'NONE',  ( 0.000000000000000000, 0.000000000000000000, -1.000000000000000000 ) ) ;
#105016=ORIENTED_EDGE ( 'NONE', *, *, #54861, .F. ) ;
#105017=LINE ( 'NONE', #55295, #115953 ) ;
#105018=CONICAL_SURFACE ( 'NONE', #27753, 0.1000000000000002554, 0.003490658503988666988 ) ;
#105019=AXIS2_PLACEMENT_3D ( 'NONE', #9762, #39886, #49707 ) ;
#105020=ORIENTED_EDGE ( 'NONE', *, *, #16223, .F. ) ;
#105022=AXIS2_PLACEMENT_3D ( 'NONE', #3914, #41286, #42579 ) ;
#105023=ORIENTED_EDGE ( 'NONE', *, *, #46638, .T. ) ;
#105024=DIRECTION ( 'NONE',  ( 0.000000000000000000, -0.9999939076577903929, 0.003490651415223739937 ) ) ;
#105025=DIRECTION ( 'NONE',  ( -0.000000000000000000, 1.000000000000000000, -0.000000000000000000 ) ) ;
#105026=AXIS2_PLACEMENT_3D ( 'NONE', #104982, #123354, #15310 ) ;
#105027=AXIS2_PLACEMENT_3D ( 'NONE', #531, #20836, #29376 ) ;
#105028=DIRECTION ( 'NONE',  ( -0.000000000000000000, -1.000000000000000000, -0.000000000000000000 ) ) ;
#105029=ADVANCED_FACE ( 'NONE', ( #76275 ), #86509, .T. ) ;
#105030=CARTESIAN_POINT ( 'NONE',  ( 9.349999999999916156, 2.500000000000000000, -1.718653347947326049 ) ) ;
#105032=AXIS2_PLACEMENT_3D ( 'NONE', #35830, #14863, #26017 ) ;
#105033=DIRECTION ( 'NONE',  ( 0.000000000000000000, 1.000000000000000000, 0.000000000000000000 ) ) ;
#105034=DIRECTION ( 'NONE',  ( 0.000000000000000000, 1.000000000000000000, 0.000000000000000000 ) ) ;
#105035=ORIENTED_EDGE ( 'NONE', *, *, #107130, .F. ) ;
#105036=VERTEX_POINT ( 'NONE', #89953 ) ;
#105037=ORIENTED_EDGE ( 'NONE', *, *, #73261, .F. ) ;
#105038=FACE_OUTER_BOUND ( 'NONE', #56509, .T. ) ;
#105039=CARTESIAN_POINT ( 'NONE',  ( -2.300000000000033129, 12.50000000000000000, 3.983716857408420076 ) ) ;
#105041=DIRECTION ( 'NONE',  ( -0.000000000000000000, 1.000000000000000000, -0.000000000000000000 ) ) ;
#105042=AXIS2_PLACEMENT_3D ( 'NONE', #123922, #2211, #33627 ) ;
#105043=DIRECTION ( 'NONE',  ( 0.000000000000000000, 0.000000000000000000, -1.000000000000000000 ) ) ;
#105044=ADVANCED_FACE ( 'NONE', ( #1570 ), #88573, .T. ) ;
#105045=CARTESIAN_POINT ( 'NONE',  ( -5.400000000000024336, 2.500000000000000000, -3.737306695894649700 ) ) ;
#105046=AXIS2_PLACEMENT_3D ( 'NONE', #120053, #21200, #29735 ) ;
#105047=ORIENTED_EDGE ( 'NONE', *, *, #24179, .T. ) ;
#105048=CARTESIAN_POINT ( 'NONE',  ( -2.700000000000030820, 2.500000000000000000, -4.083716857408426826 ) ) ;
#105049=CIRCLE ( 'NONE', #119724, 0.1000000000000002554 ) ;
#105050=EDGE_LOOP ( 'NONE', ( #116808, #48475, #13756, #27322 ) ) ;
#105051=EDGE_CURVE ( 'NONE', #33059, #39246, #19940, .T. ) ;
#105052=DIRECTION ( 'NONE',  ( -4.274815082592931898E-19, -0.9999939076577903929, -0.003490651415223739937 ) ) ;
#105053=CARTESIAN_POINT ( 'NONE',  ( 11.84999999999990727, 2.500000000000000000, 6.941600689897073018 ) ) ;
#105054=CARTESIAN_POINT ( 'NONE',  ( -9.600000000000008527, 2.500000000000000000, -4.230127018922197557 ) ) ;
#105055=AXIS2_PLACEMENT_3D ( 'NONE', #87378, #69031, #78883 ) ;
#105056=AXIS2_PLACEMENT_3D ( 'NONE', #19551, #9085, #49036 ) ;
#105057=ORIENTED_EDGE ( 'NONE', *, *, #121985, .F. ) ;
#105058=AXIS2_PLACEMENT_3D ( 'NONE', #43355, #102887, #13866 ) ;
#105059=VECTOR ( 'NONE', #34259, 1000.000000000000000 ) ;
#105060=CARTESIAN_POINT ( 'NONE',  ( 0.8499999999999553468, 12.50000000000000000, 1.472243186433545459 ) ) ;
#105062=CONICAL_SURFACE ( 'NONE', #25658, 0.09999999999999982514, 0.003490658503988666988 ) ;
#105063=VERTEX_POINT ( 'NONE', #59886 ) ;
#105064=FACE_OUTER_BOUND ( 'NONE', #29982, .T. ) ;
#105066=ORIENTED_EDGE ( 'NONE', *, *, #8470, .T. ) ;
#105067=AXIS2_PLACEMENT_3D ( 'NONE', #62219, #91660, #92298 ) ;
#105068=ORIENTED_EDGE ( 'NONE', *, *, #72619, .F. ) ;
#105069=AXIS2_PLACEMENT_3D ( 'NONE', #19686, #129022, #37401 ) ;
#105070=CARTESIAN_POINT ( 'NONE',  ( 11.64999999999990266, 2.500000000000000000, -6.395190528383301931 ) ) ;
#105071=CONICAL_SURFACE ( 'NONE', #48672, 0.09999999999999999167, 0.003490658503988666988 ) ;
#105072=ORIENTED_EDGE ( 'NONE', *, *, #49431, .F. ) ;
#105073=CARTESIAN_POINT ( 'NONE',  ( -11.44999999999999929, 2.500000000000000000, -1.818653347947322141 ) ) ;
#105075=FACE_OUTER_BOUND ( 'NONE', #75138, .T. ) ;
#105076=EDGE_LOOP ( 'NONE', ( #13222, #45391, #5641, #109313 ) ) ;
#105077=ADVANCED_FACE ( 'NONE', ( #61804 ), #42632, .T. ) ;
#105078=FACE_BOUND ( 'NONE', #98768, .T. ) ;
#105079=CIRCLE ( 'NONE', #17336, 0.06509327318403741736 ) ;
#105080=DIRECTION ( 'NONE',  ( 0.000000000000000000, 1.000000000000000000, 0.000000000000000000 ) ) ;
#105081=EDGE_LOOP ( 'NONE', ( #8686, #80109, #126954, #127880 ) ) ;
#105082=FACE_OUTER_BOUND ( 'NONE', #12033, .T. ) ;
#105083=CARTESIAN_POINT ( 'NONE',  ( -8.950000000000008171, 12.50000000000000000, -2.446380397790840266 ) ) ;
#105084=ADVANCED_FACE ( 'NONE', ( #40889 ), #48888, .T. ) ;
#105085=ORIENTED_EDGE ( 'NONE', *, *, #76588, .T. ) ;
#105086=EDGE_LOOP ( 'NONE', ( #116511, #16466 ) ) ;
#105087=ORIENTED_EDGE ( 'NONE', *, *, #8775, .T. ) ;
#105088=LINE ( 'NONE', #24622, #14799 ) ;
#105089=CARTESIAN_POINT ( 'NONE',  ( 2.500000000000002220, 2.500000000000000000, 9.000000000000005329 ) ) ;
#105090=EDGE_CURVE ( 'NONE', #99080, #55788, #80272, .T. ) ;
#105091=ADVANCED_FACE ( 'NONE', ( #110246 ), #61404, .T. ) ;
#105092=CARTESIAN_POINT ( 'NONE',  ( -7.050000000000013145, 2.500000000000000000, 2.165063509461097713 ) ) ;
#105093=AXIS2_PLACEMENT_3D ( 'NONE', #97498, #66095, #106033 ) ;
#105094=EDGE_CURVE ( 'NONE', #68510, #26528, #81438, .T. ) ;
#105095=FACE_BOUND ( 'NONE', #65620, .T. ) ;
#105096=VERTEX_POINT ( 'NONE', #50677 ) ;
#105097=ADVANCED_FACE ( 'NONE', ( #61147 ), #2903, .T. ) ;
#105099=ADVANCED_FACE ( 'NONE', ( #2208 ), #76060, .T. ) ;
#105100=CARTESIAN_POINT ( 'NONE',  ( 5.849999999999932143, 2.500000000000000000, 2.065063509461097624 ) ) ;
#105101=LINE ( 'NONE', #46852, #89905 ) ;
#105102=PLANE ( 'NONE',  #124425 ) ;
#105103=VECTOR ( 'NONE', #39322, 1000.000000000000000 ) ;
#105104=AXIS2_PLACEMENT_3D ( 'NONE', #126256, #14977, #16905 ) ;
#105105=CARTESIAN_POINT ( 'NONE',  ( 4.599999999999938360, 12.50000000000000000, -0.06509327318403970719 ) ) ;
#105106=DIRECTION ( 'NONE',  ( 0.000000000000000000, 1.000000000000000000, 0.000000000000000000 ) ) ;
#105107=EDGE_CURVE ( 'NONE', #37993, #26037, #19627, .T. ) ;
#105108=CARTESIAN_POINT ( 'NONE',  ( -4.121192902244064579E-14, 2.500000000000000000, 3.537306695894645081 ) ) ;
#105109=LINE ( 'NONE', #37683, #113041 ) ;
#105110=EDGE_CURVE ( 'NONE', #23819, #40507, #11395, .T. ) ;
#105111=VECTOR ( 'NONE', #76550, 1000.000000000000000 ) ;
#105112=ADVANCED_FACE ( 'NONE', ( #32366 ), #103253, .T. ) ;
#105113=VECTOR ( 'NONE', #56743, 1000.000000000000000 ) ;
#105115=VECTOR ( 'NONE', #117422, 1000.000000000000000 ) ;
#105116=ORIENTED_EDGE ( 'NONE', *, *, #23123, .T. ) ;
#105117=ORIENTED_EDGE ( 'NONE', *, *, #126318, .T. ) ;
#105118=EDGE_LOOP ( 'NONE', ( #87634, #70997, #38066, #95164 ) ) ;
#105119=ORIENTED_EDGE ( 'NONE', *, *, #72546, .F. ) ;
#105120=AXIS2_PLACEMENT_3D ( 'NONE', #91808, #100346, #51261 ) ;
#105121=EDGE_LOOP ( 'NONE', ( #126544, #122869, #104927, #81954 ) ) ;
#105122=DIRECTION ( 'NONE',  ( -4.274815082592931898E-19, -0.9999939076577903929, -0.003490651415223739937 ) ) ;
#105123=VECTOR ( 'NONE', #10749, 1000.000000000000000 ) ;
#105124=DIRECTION ( 'NONE',  ( 0.000000000000000000, 0.000000000000000000, 1.000000000000000000 ) ) ;
#105125=ORIENTED_EDGE ( 'NONE', *, *, #76880, .F. ) ;
#105126=FACE_BOUND ( 'NONE', #56699, .T. ) ;
#105127=CIRCLE ( 'NONE', #65319, 0.09999999999999982514 ) ;
#105128=DIRECTION ( 'NONE',  ( -0.000000000000000000, -1.000000000000000000, -0.000000000000000000 ) ) ;
#105129=LINE ( 'NONE', #107057, #38587 ) ;
#105130=VERTEX_POINT ( 'NONE', #19264 ) ;
#105131=CARTESIAN_POINT ( 'NONE',  ( 8.349999999999923261, 2.500000000000000000, -5.702370205355749455 ) ) ;
#105132=CARTESIAN_POINT ( 'NONE',  ( -3.750000000000025757, 2.500000000000000000, 1.472243186433545459 ) ) ;
#105133=PLANE ( 'NONE',  #45460 ) ;
#105134=ORIENTED_EDGE ( 'NONE', *, *, #87652, .F. ) ;
#105135=PLANE ( 'NONE',  #99380 ) ;
#105136=CIRCLE ( 'NONE', #31904, 0.1000000000000002554 ) ;
#105137=ORIENTED_EDGE ( 'NONE', *, *, #92396, .F. ) ;
#105138=ORIENTED_EDGE ( 'NONE', *, *, #32601, .T. ) ;
#105139=ORIENTED_EDGE ( 'NONE', *, *, #85301, .F. ) ;
#105140=DIRECTION ( 'NONE',  ( 0.000000000000000000, 1.000000000000000000, 0.000000000000000000 ) ) ;
#105141=DIRECTION ( 'NONE',  ( -0.000000000000000000, 1.000000000000000000, -0.000000000000000000 ) ) ;
#105142=DIRECTION ( 'NONE',  ( 0.000000000000000000, 1.000000000000000000, 0.000000000000000000 ) ) ;
#105143=VERTEX_POINT ( 'NONE', #59235 ) ;
#105144=CARTESIAN_POINT ( 'NONE',  ( 12.64862127202694353, 1.500000000000319300, -8.430718248283330496 ) ) ;
#105145=CONICAL_SURFACE ( 'NONE', #94685, 0.1000000000000000472, 0.003490658503988666988 ) ;
#105146=DIRECTION ( 'NONE',  ( 0.000000000000000000, 1.000000000000000000, 0.000000000000000000 ) ) ;
#105147=ADVANCED_FACE ( 'NONE', ( #9469 ), #89316, .T. ) ;
#105148=CARTESIAN_POINT ( 'NONE',  ( -0.6500000000000394351, 2.500000000000000000, 2.511473670974873507 ) ) ;
#105150=CARTESIAN_POINT ( 'NONE',  ( -6.450000000000016165, 12.50000000000000000, 6.776507416713035248 ) ) ;
#105151=CARTESIAN_POINT ( 'NONE',  ( -4.600000000000024514, 12.50000000000000000, -0.6928203230275542523 ) ) ;
#105152=EDGE_CURVE ( 'NONE', #115126, #18421, #119400, .T. ) ;
#105153=AXIS2_PLACEMENT_3D ( 'NONE', #47161, #86422, #75961 ) ;
#105154=ORIENTED_EDGE ( 'NONE', *, *, #73771, .F. ) ;
#105155=DIRECTION ( 'NONE',  ( -0.000000000000000000, -1.000000000000000000, -0.000000000000000000 ) ) ;
#105156=CONICAL_SURFACE ( 'NONE', #73864, 0.1000000000000002554, 0.003490658503988666988 ) ;
#105157=EDGE_CURVE ( 'NONE', #11967, #29091, #839, .T. ) ;
#105158=CIRCLE ( 'NONE', #113475, 0.06509327318403745899 ) ;
#105159=ORIENTED_EDGE ( 'NONE', *, *, #55855, .T. ) ;
#105160=CIRCLE ( 'NONE', #121895, 0.1000000000000000472 ) ;
#105161=ADVANCED_FACE ( 'NONE', ( #20582 ), #84370, .T. ) ;
#105162=EDGE_LOOP ( 'NONE', ( #65122, #115317 ) ) ;
#105163=DIRECTION ( 'NONE',  ( 0.000000000000000000, 0.000000000000000000, -1.000000000000000000 ) ) ;
#105164=FACE_OUTER_BOUND ( 'NONE', #83310, .T. ) ;
#105165=CARTESIAN_POINT ( 'NONE',  ( 4.349999999999937472, 2.500000000000000000, 6.841600689897072485 ) ) ;
#105166=CARTESIAN_POINT ( 'NONE',  ( -2.300000000000033573, 2.500000000000000000, -3.983716857408426293 ) ) ;
#105167=DIRECTION ( 'NONE',  ( 0.000000000000000000, 0.000000000000000000, 1.000000000000000000 ) ) ;
#105168=CIRCLE ( 'NONE', #15260, 0.06509327318403745899 ) ;
#105169=ORIENTED_EDGE ( 'NONE', *, *, #79140, .F. ) ;
#105170=EDGE_CURVE ( 'NONE', #101388, #86861, #74004, .T. ) ;
#105171=ORIENTED_EDGE ( 'NONE', *, *, #49242, .T. ) ;
#105172=CARTESIAN_POINT ( 'NONE',  ( -3.750000000000027534, 12.50000000000000000, -1.407149913249512663 ) ) ;
#105173=DIRECTION ( 'NONE',  ( -0.000000000000000000, 1.000000000000000000, -0.000000000000000000 ) ) ;
#105174=AXIS2_PLACEMENT_3D ( 'NONE', #32624, #111120, #81683 ) ;
#105175=VECTOR ( 'NONE', #67684, 1000.000000000000000 ) ;
#105176=AXIS2_PLACEMENT_3D ( 'NONE', #120309, #72505, #40475 ) ;
#105177=DIRECTION ( 'NONE',  ( 0.000000000000000000, -0.000000000000000000, 1.000000000000000000 ) ) ;
#105178=ORIENTED_EDGE ( 'NONE', *, *, #11414, .T. ) ;
#105179=EDGE_LOOP ( 'NONE', ( #108745, #61698 ) ) ;
#105180=DIRECTION ( 'NONE',  ( 0.000000000000000000, 0.000000000000000000, 1.000000000000000000 ) ) ;
#105181=CIRCLE ( 'NONE', #622, 0.09999999999999999167 ) ;
#105182=ORIENTED_EDGE ( 'NONE', *, *, #109896, .F. ) ;
#105183=DIRECTION ( 'NONE',  ( -4.274815082592931898E-19, -0.9999939076577903929, -0.003490651415223739937 ) ) ;
#105184=CARTESIAN_POINT ( 'NONE',  ( -13.74999999999998934, 2.500000000000000000, -1.472243186433547901 ) ) ;
#105185=ORIENTED_EDGE ( 'NONE', *, *, #108587, .T. ) ;
#105186=AXIS2_PLACEMENT_3D ( 'NONE', #110783, #81345, #33537 ) ;
#105187=FACE_OUTER_BOUND ( 'NONE', #91921, .T. ) ;
#105188=DIRECTION ( 'NONE',  ( -0.000000000000000000, 1.000000000000000000, -0.000000000000000000 ) ) ;
#105189=FACE_OUTER_BOUND ( 'NONE', #14020, .T. ) ;
#105190=EDGE_CURVE ( 'NONE', #5028, #4651, #50939, .T. ) ;
#105191=CARTESIAN_POINT ( 'NONE',  ( -4.150000000000025224, 12.50000000000000000, 5.802370205355744659 ) ) ;
#105192=ORIENTED_EDGE ( 'NONE', *, *, #118368, .F. ) ;
#105193=DIRECTION ( 'NONE',  ( 0.000000000000000000, 0.000000000000000000, -1.000000000000000000 ) ) ;
#105194=DIRECTION ( 'NONE',  ( 0.000000000000000000, 0.000000000000000000, 1.000000000000000000 ) ) ;
#105195=EDGE_LOOP ( 'NONE', ( #46572, #89987, #15232, #95999 ) ) ;
#105196=EDGE_LOOP ( 'NONE', ( #47694, #99727, #86317, #51428 ) ) ;
#105197=CIRCLE ( 'NONE', #126129, 0.06509327318403745899 ) ;
#105198=CONICAL_SURFACE ( 'NONE', #92684, 0.1000000000000002554, 0.003490658503988666988 ) ;
#105199=DIRECTION ( 'NONE',  ( 0.000000000000000000, 1.000000000000000000, 0.000000000000000000 ) ) ;
#105200=DIRECTION ( 'NONE',  ( -0.000000000000000000, 1.000000000000000000, -0.000000000000000000 ) ) ;
#105201=DIRECTION ( 'NONE',  ( 0.000000000000000000, 1.000000000000000000, 0.000000000000000000 ) ) ;
#105202=FACE_OUTER_BOUND ( 'NONE', #1968, .T. ) ;
#105203=CARTESIAN_POINT ( 'NONE',  ( 8.099999999999921485, 12.50000000000000000, 0.3464101615137735735 ) ) ;
#105204=DIRECTION ( 'NONE',  ( 0.000000000000000000, 0.000000000000000000, 1.000000000000000000 ) ) ;
#105205=VECTOR ( 'NONE', #97836, 1000.000000000000000 ) ;
#105206=DIRECTION ( 'NONE',  ( 0.000000000000000000, 0.000000000000000000, -1.000000000000000000 ) ) ;
#105207=EDGE_CURVE ( 'NONE', #55907, #24394, #63730, .T. ) ;
#105208=AXIS2_PLACEMENT_3D ( 'NONE', #47674, #88199, #56813 ) ;
#105209=FACE_OUTER_BOUND ( 'NONE', #62696, .T. ) ;
#105210=DIRECTION ( 'NONE',  ( 0.000000000000000000, 0.000000000000000000, -1.000000000000000000 ) ) ;
#105211=DIRECTION ( 'NONE',  ( -0.000000000000000000, -1.000000000000000000, -0.000000000000000000 ) ) ;
#105212=VECTOR ( 'NONE', #69251, 1000.000000000000000 ) ;
#105213=CIRCLE ( 'NONE', #107353, 0.06509327318403741736 ) ;
#105214=DIRECTION ( 'NONE',  ( 0.000000000000000000, 0.000000000000000000, 1.000000000000000000 ) ) ;
#105215=EDGE_LOOP ( 'NONE', ( #34892, #62992 ) ) ;
#105216=VECTOR ( 'NONE', #124402, 1000.000000000000000 ) ;
#105217=AXIS2_PLACEMENT_3D ( 'NONE', #110173, #20506, #49981 ) ;
#105218=AXIS2_PLACEMENT_3D ( 'NONE', #62424, #51322, #111497 ) ;
#105219=ORIENTED_EDGE ( 'NONE', *, *, #65699, .T. ) ;
#105220=VECTOR ( 'NONE', #84231, 1000.000000000000000 ) ;
#105221=CONICAL_SURFACE ( 'NONE', #50851, 0.1000000000000002554, 0.003490658503988666988 ) ;
#105222=ORIENTED_EDGE ( 'NONE', *, *, #82567, .T. ) ;
#105223=EDGE_CURVE ( 'NONE', #42007, #16778, #14599, .T. ) ;
#105224=CARTESIAN_POINT ( 'NONE',  ( 5.449999999999934452, 2.500000000000000000, 2.065063509461097624 ) ) ;
#105225=DIRECTION ( 'NONE',  ( 0.000000000000000000, 1.000000000000000000, 0.000000000000000000 ) ) ;
#105226=CARTESIAN_POINT ( 'NONE',  ( 6.649999999999930189, 12.50000000000000000, 5.802370205355744659 ) ) ;
#105227=EDGE_LOOP ( 'NONE', ( #1161, #86384 ) ) ;
#105228=DIRECTION ( 'NONE',  ( -0.000000000000000000, -1.000000000000000000, -0.000000000000000000 ) ) ;
#105229=FACE_OUTER_BOUND ( 'NONE', #116851, .T. ) ;
#105230=DIRECTION ( 'NONE',  ( 0.000000000000000000, 1.000000000000000000, 0.000000000000000000 ) ) ;
#105231=EDGE_LOOP ( 'NONE', ( #92528, #332 ) ) ;
#105232=( BOUNDED_SURFACE ( )  B_SPLINE_SURFACE ( 3, 2, ( 
 ( #43002, #40410, #92057 ),
 ( #60057, #2369, #42328 ),
 ( #22057, #3054, #20751 ),
 ( #52782, #90114, #92717 ),
 ( #61970, #1740, #60692 ),
 ( #31231, #122184, #50861 ),
 ( #101893, #82260, #112358 ),
 ( #82903, #71132, #72436 ),
 ( #22703, #122822, #51510 ),
 ( #62624, #99962, #12833 ),
 ( #33165, #80327, #73074 ),
 ( #100587, #10290, #50228 ),
 ( #443, #1103, #120251 ),
 ( #70492, #110415, #41062 ),
 ( #101244, #80967, #120879 ),
 ( #111037, #21388, #61328 ),
 ( #91424, #41698, #105759 ),
 ( #65816, #14761, #4297 ),
 ( #125397, #33789, #83547 ),
 ( #105089, #114913, #85464 ) ),
 .UNSPECIFIED., .F., .F., .F. ) 
 B_SPLINE_SURFACE_WITH_KNOTS ( ( 4, 2, 2, 2, 2, 2, 2, 2, 2, 4 ),
 ( 3, 3 ),
 ( 5.475220971051797392E-18, 0.0008832438798941970272, 0.001766487759788388633, 0.002649731639682580131, 0.003532975519576771629, 0.005299463279365155058, 0.007065951039153538053, 0.008832438798941921049, 0.01059892655873030491, 0.01413190207830707090 ),
 ( 0.000000000000000000, 1.000000000000000000 ),
 .UNSPECIFIED. ) 
 GEOMETRIC_REPRESENTATION_ITEM ( )  RATIONAL_B_SPLINE_SURFACE ( (
 ( 1.000000000000000000, 0.7071067811865472397, 1.000000000000000000),
 ( 1.000000000000000000, 0.7071067811865472397, 1.000000000000000000),
 ( 1.000000000000000000, 0.7071067811865476838, 1.000000000000000000),
 ( 1.000000000000000000, 0.7071067811865476838, 1.000000000000000000),
 ( 1.000000000000000000, 0.7071067811865471286, 1.000000000000000000),
 ( 1.000000000000000000, 0.7071067811865471286, 1.000000000000000000),
 ( 1.000000000000000000, 0.7071067811865471286, 1.000000000000000000),
 ( 1.000000000000000000, 0.7071067811865471286, 1.000000000000000000),
 ( 1.000000000000000000, 0.7071067811865476838, 1.000000000000000000),
 ( 1.000000000000000000, 0.7071067811865476838, 1.000000000000000000),
 ( 1.000000000000000000, 0.7071067811865476838, 1.000000000000000000),
 ( 1.000000000000000000, 0.7071067811865476838, 1.000000000000000000),
 ( 1.000000000000000000, 0.7071067811865473507, 1.000000000000000000),
 ( 1.000000000000000000, 0.7071067811865473507, 1.000000000000000000),
 ( 1.000000000000000000, 0.7071067811865473507, 1.000000000000000000),
 ( 1.000000000000000000, 0.7071067811865473507, 1.000000000000000000),
 ( 1.000000000000000000, 0.7071067811865479058, 1.000000000000000000),
 ( 1.000000000000000000, 0.7071067811865479058, 1.000000000000000000),
 ( 1.000000000000000000, 0.7071067811865473507, 1.000000000000000000),
 ( 1.000000000000000000, 0.7071067811865473507, 1.000000000000000000) ) ) 
 REPRESENTATION_ITEM ( '' )  SURFACE ( )  );
#105233=AXIS2_PLACEMENT_3D ( 'NONE', #46031, #85922, #125855 ) ;
#105234=FACE_OUTER_BOUND ( 'NONE', #117814, .T. ) ;
#105235=ORIENTED_EDGE ( 'NONE', *, *, #21395, .T. ) ;
#105236=EDGE_CURVE ( 'NONE', #71030, #120080, #9156, .T. ) ;
#105237=ORIENTED_EDGE ( 'NONE', *, *, #128287, .T. ) ;
#105238=ORIENTED_EDGE ( 'NONE', *, *, #18256, .T. ) ;
#105239=ORIENTED_EDGE ( 'NONE', *, *, #112845, .F. ) ;
#105240=DIRECTION ( 'NONE',  ( 0.000000000000000000, 0.000000000000000000, 1.000000000000000000 ) ) ;
#105241=CARTESIAN_POINT ( 'NONE',  ( 10.19999999999991047, 12.50000000000000000, 4.676537180435972552 ) ) ;
#105242=AXIS2_PLACEMENT_3D ( 'NONE', #125523, #123585, #64671 ) ;
#105243=DIRECTION ( 'NONE',  ( -0.000000000000000000, 1.000000000000000000, -0.000000000000000000 ) ) ;
#105244=CIRCLE ( 'NONE', #59303, 0.06509327318403745899 ) ;
#105245=CARTESIAN_POINT ( 'NONE',  ( -8.950000000000004619, 2.500000000000000000, 6.148780366869520897 ) ) ;
#105246=CIRCLE ( 'NONE', #111506, 0.06509327318403745899 ) ;
#105247=EDGE_LOOP ( 'NONE', ( #76859, #88414, #5591, #5361 ) ) ;
#105248=EDGE_CURVE ( 'NONE', #26576, #75844, #112182, .T. ) ;
#105249=CARTESIAN_POINT ( 'NONE',  ( 11.24999999999991118, 12.50000000000000000, -2.857883832488653741 ) ) ;
#105250=ORIENTED_EDGE ( 'NONE', *, *, #32810, .F. ) ;
#105251=CARTESIAN_POINT ( 'NONE',  ( 43.31214921624317071, -3.511364963957428031, -3.941696051812598078 ) ) ;
#105252=DIRECTION ( 'NONE',  ( 0.000000000000000000, 0.000000000000000000, 1.000000000000000000 ) ) ;
#105253=CARTESIAN_POINT ( 'NONE',  ( -13.34999999999999076, 12.50000000000000000, 2.099970236277064028 ) ) ;
#105254=CARTESIAN_POINT ( 'NONE',  ( 17.33812564108897902, -2.538896947917432811, 5.379288978441534752 ) ) ;
#105255=CIRCLE ( 'NONE', #48842, 0.06509327318403745899 ) ;
#105256=EDGE_CURVE ( 'NONE', #21947, #119719, #78121, .T. ) ;
#105257=VERTEX_POINT ( 'NONE', #72903 ) ;
#105258=CIRCLE ( 'NONE', #65549, 0.09999999999999982514 ) ;
#105259=EDGE_LOOP ( 'NONE', ( #82764, #101132, #22539, #58948 ) ) ;
#105260=VERTEX_POINT ( 'NONE', #83372 ) ;
#105261=FACE_OUTER_BOUND ( 'NONE', #68493, .T. ) ;
#105262=CARTESIAN_POINT ( 'NONE',  ( -6.450000000000014388, 12.50000000000000000, 1.818653347947321475 ) ) ;
#105263=ADVANCED_FACE ( 'NONE', ( #104909 ), #21689, .T. ) ;
#105264=ADVANCED_FACE ( 'NONE', ( #4133 ), #13319, .T. ) ;
#105265=DIRECTION ( 'NONE',  ( -0.000000000000000000, -1.000000000000000000, -0.000000000000000000 ) ) ;
#105266=EDGE_CURVE ( 'NONE', #77033, #36233, #3516, .T. ) ;
#105267=FACE_BOUND ( 'NONE', #127064, .T. ) ;
#105268=AXIS2_PLACEMENT_3D ( 'NONE', #122868, #32574, #100165 ) ;
#105269=ADVANCED_FACE ( 'NONE', ( #43458 ), #34218, .T. ) ;
#105270=CARTESIAN_POINT ( 'NONE',  ( -3.150000000000033218, 2.500000000000000000, -6.841600689897078702 ) ) ;
#105271=LINE ( 'NONE', #8348, #90492 ) ;
#105272=CARTESIAN_POINT ( 'NONE',  ( 3.149999999999944400, 12.50000000000000000, 1.753560074763284016 ) ) ;
#105273=FACE_OUTER_BOUND ( 'NONE', #6451, .T. ) ;
#105274=CIRCLE ( 'NONE', #29978, 0.1000000000000000472 ) ;
#105275=AXIS2_PLACEMENT_3D ( 'NONE', #10470, #120438, #77922 ) ;
#105276=EDGE_CURVE ( 'NONE', #53613, #34661, #32165, .T. ) ;
#105277=CARTESIAN_POINT ( 'NONE',  ( -8.950000000000011724, 2.500000000000000000, -6.048780366869521252 ) ) ;
#105278=EDGE_CURVE ( 'NONE', #95476, #75694, #105303, .T. ) ;
#105280=AXIS2_PLACEMENT_3D ( 'NONE', #57976, #97884, #68423 ) ;
#105281=EDGE_CURVE ( 'NONE', #14873, #11223, #40672, .T. ) ;
#105282=DIRECTION ( 'NONE',  ( 0.000000000000000000, 0.000000000000000000, -1.000000000000000000 ) ) ;
#105283=CIRCLE ( 'NONE', #107429, 0.1000000000000002554 ) ;
#105284=EDGE_CURVE ( 'NONE', #110245, #89903, #84469, .T. ) ;
#105285=ADVANCED_FACE ( 'NONE', ( #102367 ), #80367, .T. ) ;
#105286=FACE_OUTER_BOUND ( 'NONE', #122840, .T. ) ;
#105287=ORIENTED_EDGE ( 'NONE', *, *, #122850, .F. ) ;
#105288=ORIENTED_EDGE ( 'NONE', *, *, #94437, .F. ) ;
#105289=VERTEX_POINT ( 'NONE', #73525 ) ;
#105290=EDGE_LOOP ( 'NONE', ( #116779, #35286 ) ) ;
#105291=DIRECTION ( 'NONE',  ( 0.000000000000000000, 0.000000000000000000, -1.000000000000000000 ) ) ;
#105292=FACE_BOUND ( 'NONE', #4175, .T. ) ;
#105293=ADVANCED_FACE ( 'NONE', ( #4775 ), #57371, .T. ) ;
#105294=DIRECTION ( 'NONE',  ( -4.274815082592931898E-19, -0.9999939076577903929, -0.003490651415223739937 ) ) ;
#105295=CIRCLE ( 'NONE', #96976, 0.09999999999999999167 ) ;
#105296=ORIENTED_EDGE ( 'NONE', *, *, #102441, .T. ) ;
#105297=CARTESIAN_POINT ( 'NONE',  ( 59.74180401152909781, 3.401974578027094243, 5.439313020113218045 ) ) ;
#105298=AXIS2_PLACEMENT_3D ( 'NONE', #52339, #81787, #51073 ) ;
#105299=DIRECTION ( 'NONE',  ( -0.000000000000000000, -1.000000000000000000, -0.000000000000000000 ) ) ;
#105301=DIRECTION ( 'NONE',  ( 0.000000000000000000, 1.000000000000000000, 0.000000000000000000 ) ) ;
#105302=DIRECTION ( 'NONE',  ( 0.000000000000000000, 0.000000000000000000, 1.000000000000000000 ) ) ;
#105303=CIRCLE ( 'NONE', #117901, 0.1000000000000002554 ) ;
#105304=AXIS2_PLACEMENT_3D ( 'NONE', #16800, #56725, #18760 ) ;
#105305=CIRCLE ( 'NONE', #109416, 0.1000000000000000472 ) ;
#105306=CIRCLE ( 'NONE', #743, 0.1000000000000002554 ) ;
#105307=AXIS2_PLACEMENT_3D ( 'NONE', #77374, #117259, #38093 ) ;
#105308=ORIENTED_EDGE ( 'NONE', *, *, #113819, .F. ) ;
#105309=CARTESIAN_POINT ( 'NONE',  ( 1.899999999999949507, 12.50000000000000000, 3.983716857408420964 ) ) ;
#105310=CARTESIAN_POINT ( 'NONE',  ( 2.099999999999950351, 2.500000000000000000, -0.5928203230275541635 ) ) ;
#105311=AXIS2_PLACEMENT_3D ( 'NONE', #12344, #22840, #20245 ) ;
#105312=VECTOR ( 'NONE', #37416, 1000.000000000000000 ) ;
#105313=ORIENTED_EDGE ( 'NONE', *, *, #36439, .T. ) ;
#105314=VECTOR ( 'NONE', #45411, 1000.000000000000000 ) ;
#105315=CARTESIAN_POINT ( 'NONE',  ( -7.500000000000015099, 2.500000000000000000, -5.022947341949754119 ) ) ;
#105316=CARTESIAN_POINT ( 'NONE',  ( 13.09999999999990195, 2.500000000000000000, -4.576537180435978236 ) ) ;
#105317=LINE ( 'NONE', #35925, #11697 ) ;
#105318=AXIS2_PLACEMENT_3D ( 'NONE', #113245, #45171, #102772 ) ;
#105319=ORIENTED_EDGE ( 'NONE', *, *, #16278, .T. ) ;
#105320=ORIENTED_EDGE ( 'NONE', *, *, #15389, .F. ) ;
#105321=DIRECTION ( 'NONE',  ( -0.000000000000000000, 1.000000000000000000, -0.000000000000000000 ) ) ;
#105322=VERTEX_POINT ( 'NONE', #2873 ) ;
#105323=CARTESIAN_POINT ( 'NONE',  ( 6.649999999999930189, 2.500000000000000000, 7.188010851410848723 ) ) ;
#105324=CARTESIAN_POINT ( 'NONE',  ( 4.399999999999940847, 2.500000000000000000, -3.883716857408426648 ) ) ;
#105325=EDGE_CURVE ( 'NONE', #25509, #92080, #82738, .T. ) ;
#105326=ORIENTED_EDGE ( 'NONE', *, *, #115710, .F. ) ;
#105327=DIRECTION ( 'NONE',  ( 0.000000000000000000, 1.000000000000000000, 0.000000000000000000 ) ) ;
#105328=EDGE_CURVE ( 'NONE', #35395, #103698, #101199, .T. ) ;
#105329=DIRECTION ( 'NONE',  ( 0.000000000000000000, -0.9999939076577903929, 0.003490651415223739937 ) ) ;
#105330=CARTESIAN_POINT ( 'NONE',  ( -7.100000000000017408, 2.500000000000000000, -0.7928203230275543412 ) ) ;
#105331=DIRECTION ( 'NONE',  ( 0.000000000000000000, 1.000000000000000000, 0.000000000000000000 ) ) ;
#105332=DIRECTION ( 'NONE',  ( 0.000000000000000000, -0.000000000000000000, 1.000000000000000000 ) ) ;
#105333=CIRCLE ( 'NONE', #27966, 0.1000000000000000056 ) ;
#105334=EDGE_CURVE ( 'NONE', #112676, #92091, #82432, .T. ) ;
#105335=ORIENTED_EDGE ( 'NONE', *, *, #64653, .F. ) ;
#105336=ORIENTED_EDGE ( 'NONE', *, *, #27251, .F. ) ;
#105337=DIRECTION ( 'NONE',  ( 0.000000000000000000, -0.000000000000000000, 1.000000000000000000 ) ) ;
#105338=ADVANCED_FACE ( 'NONE', ( #47309 ), #90815, .T. ) ;
#105339=DIRECTION ( 'NONE',  ( 0.000000000000000000, -0.000000000000000000, 1.000000000000000000 ) ) ;
#105340=DIRECTION ( 'NONE',  ( 0.000000000000000000, 0.000000000000000000, -1.000000000000000000 ) ) ;
#105341=ORIENTED_EDGE ( 'NONE', *, *, #30969, .F. ) ;
#105342=ORIENTED_EDGE ( 'NONE', *, *, #8226, .T. ) ;
#105343=EDGE_LOOP ( 'NONE', ( #116208, #55890 ) ) ;
#105344=DIRECTION ( 'NONE',  ( 0.000000000000000000, 0.000000000000000000, 1.000000000000000000 ) ) ;
#105345=CIRCLE ( 'NONE', #40619, 0.06509327318403745899 ) ;
#105346=DIRECTION ( 'NONE',  ( 0.000000000000000000, 1.000000000000000000, 0.000000000000000000 ) ) ;
#105347=CARTESIAN_POINT ( 'NONE',  ( 3.949999999999942446, 12.50000000000000000, -6.841600689897078702 ) ) ;
#105349=DIRECTION ( 'NONE',  ( 0.000000000000000000, 0.000000000000000000, 1.000000000000000000 ) ) ;
#105350=DIRECTION ( 'NONE',  ( -0.000000000000000000, -1.000000000000000000, -0.000000000000000000 ) ) ;
#105351=DIRECTION ( 'NONE',  ( 0.000000000000000000, -0.9999939076577903929, 0.003490651415223739937 ) ) ;
#105352=DIRECTION ( 'NONE',  ( 0.000000000000000000, 0.000000000000000000, 1.000000000000000000 ) ) ;
#105353=CARTESIAN_POINT ( 'NONE',  ( 3.749999999999978684, 2.500000000000000000, -2.165063509461101710 ) ) ;
#105354=VECTOR ( 'NONE', #68565, 1000.000000000000000 ) ;
#105355=FACE_OUTER_BOUND ( 'NONE', #118242, .T. ) ;
#105356=AXIS2_PLACEMENT_3D ( 'NONE', #64434, #63806, #24521 ) ;
#105357=ORIENTED_EDGE ( 'NONE', *, *, #17757, .T. ) ;
#105358=CONICAL_SURFACE ( 'NONE', #119931, 0.1000000000000002554, 0.003490658503988666988 ) ;
#105359=DIRECTION ( 'NONE',  ( 0.000000000000000000, 0.000000000000000000, 1.000000000000000000 ) ) ;
#105360=ORIENTED_EDGE ( 'NONE', *, *, #79134, .T. ) ;
#105362=DIRECTION ( 'NONE',  ( -0.000000000000000000, -1.000000000000000000, -0.000000000000000000 ) ) ;
#105363=CARTESIAN_POINT ( 'NONE',  ( 8.349999999999923261, 12.50000000000000000, -6.560283801567339701 ) ) ;
#105364=PLANE ( 'NONE',  #128021 ) ;
#105365=ADVANCED_FACE ( 'NONE', ( #55832 ), #5030, .T. ) ;
#105367=CARTESIAN_POINT ( 'NONE',  ( 0.8499999999999545697, 12.50000000000000000, 2.857883832488649301 ) ) ;
#105368=AXIS2_PLACEMENT_3D ( 'NONE', #124590, #65656, #64368 ) ;
#105369=DIRECTION ( 'NONE',  ( 0.000000000000000000, 0.000000000000000000, -1.000000000000000000 ) ) ;
#105370=AXIS2_PLACEMENT_3D ( 'NONE', #112786, #110205, #11355 ) ;
#105371=DIRECTION ( 'NONE',  ( 0.000000000000000000, 1.000000000000000000, 0.000000000000000000 ) ) ;
#105372=ORIENTED_EDGE ( 'NONE', *, *, #25234, .T. ) ;
#105373=CARTESIAN_POINT ( 'NONE',  ( -5.650000000000023448, 2.500000000000000000, -6.741600689897078169 ) ) ;
#105374=VECTOR ( 'NONE', #102410, 1000.000000000000000 ) ;
#105375=AXIS2_PLACEMENT_3D ( 'NONE', #98023, #19462, #128809 ) ;
#105376=CARTESIAN_POINT ( 'NONE',  ( 8.099999999999921485, 2.500000000000000000, -0.4464101615137783252 ) ) ;
#105377=ORIENTED_EDGE ( 'NONE', *, *, #105572, .T. ) ;
#105378=ORIENTED_EDGE ( 'NONE', *, *, #50410, .T. ) ;
#105379=EDGE_LOOP ( 'NONE', ( #91545, #74477, #11650, #12735 ) ) ;
#105380=EDGE_CURVE ( 'NONE', #39516, #58339, #78216, .T. ) ;
#105381=EDGE_CURVE ( 'NONE', #98489, #105260, #94935, .T. ) ;
#105382=EDGE_LOOP ( 'NONE', ( #14516, #64980 ) ) ;
#105384=DIRECTION ( 'NONE',  ( 0.000000000000000000, 0.000000000000000000, -1.000000000000000000 ) ) ;
#105385=CARTESIAN_POINT ( 'NONE',  ( -10.60000000000000142, 2.500000000000000000, 0.4464101615137736623 ) ) ;
#105386=DIRECTION ( 'NONE',  ( 0.000000000000000000, 1.000000000000000000, 0.000000000000000000 ) ) ;
#105387=AXIS2_PLACEMENT_3D ( 'NONE', #120987, #106800, #17103 ) ;
#105388=DIRECTION ( 'NONE',  ( -0.000000000000000000, 1.000000000000000000, -0.000000000000000000 ) ) ;
#105389=EDGE_LOOP ( 'NONE', ( #89362, #38358, #16002, #94818 ) ) ;
#105390=DIRECTION ( 'NONE',  ( 0.000000000000000000, 0.000000000000000000, 1.000000000000000000 ) ) ;
#105391=AXIS2_PLACEMENT_3D ( 'NONE', #23246, #12134, #51451 ) ;
#105392=AXIS2_PLACEMENT_3D ( 'NONE', #112409, #122235, #11617 ) ;
#105393=ADVANCED_FACE ( 'NONE', ( #127794 ), #15495, .T. ) ;
#105394=LINE ( 'NONE', #83810, #41116 ) ;
#105395=FACE_OUTER_BOUND ( 'NONE', #48707, .T. ) ;
#105396=ORIENTED_EDGE ( 'NONE', *, *, #123153, .T. ) ;
#105397=CONICAL_SURFACE ( 'NONE', #86601, 0.09999999999999982514, 0.003490658503988666988 ) ;
#105398=VECTOR ( 'NONE', #4907, 1000.000000000000000 ) ;
#105400=EDGE_LOOP ( 'NONE', ( #57581, #92267, #60811, #43277 ) ) ;
#105401=CIRCLE ( 'NONE', #48980, 0.1000000000000002554 ) ;
#105402=ORIENTED_EDGE ( 'NONE', *, *, #69082, .T. ) ;
#105403=CARTESIAN_POINT ( 'NONE',  ( 11.44999999999990870, 2.500000000000000000, -1.918653347947326004 ) ) ;
#105404=DIRECTION ( 'NONE',  ( 0.000000000000000000, 0.000000000000000000, -1.000000000000000000 ) ) ;
#105405=DIRECTION ( 'NONE',  ( 0.000000000000000000, 1.000000000000000000, 0.000000000000000000 ) ) ;
#105406=CONICAL_SURFACE ( 'NONE', #15505, 0.09999999999999982514, 0.003490658503988666988 ) ;
#105407=AXIS2_PLACEMENT_3D ( 'NONE', #110516, #60779, #100681 ) ;
#105408=AXIS2_PLACEMENT_3D ( 'NONE', #113330, #4017, #92399 ) ;
#105409=AXIS2_PLACEMENT_3D ( 'NONE', #83651, #64641, #12316 ) ;
#105410=EDGE_LOOP ( 'NONE', ( #88941, #76164 ) ) ;
#105411=DIRECTION ( 'NONE',  ( 0.000000000000000000, 0.000000000000000000, 1.000000000000000000 ) ) ;
#105412=CARTESIAN_POINT ( 'NONE',  ( 9.349999999999919709, 12.50000000000000000, 1.753560074763284016 ) ) ;
#105413=DIRECTION ( 'NONE',  ( -0.000000000000000000, 1.000000000000000000, -0.000000000000000000 ) ) ;
#105414=DIRECTION ( 'NONE',  ( 0.000000000000000000, 0.000000000000000000, 1.000000000000000000 ) ) ;
#105415=DIRECTION ( 'NONE',  ( 0.000000000000000000, 1.000000000000000000, 0.000000000000000000 ) ) ;
#105416=EDGE_CURVE ( 'NONE', #10677, #30501, #36209, .T. ) ;
#105417=VERTEX_POINT ( 'NONE', #46028 ) ;
#105418=DIRECTION ( 'NONE',  ( 0.000000000000000000, 0.000000000000000000, 1.000000000000000000 ) ) ;
#105419=ORIENTED_EDGE ( 'NONE', *, *, #36444, .T. ) ;
#105420=ORIENTED_EDGE ( 'NONE', *, *, #16789, .F. ) ;
#105421=ORIENTED_EDGE ( 'NONE', *, *, #126202, .F. ) ;
#105422=EDGE_CURVE ( 'NONE', #7810, #72282, #76768, .T. ) ;
#105423=DIRECTION ( 'NONE',  ( 0.000000000000000000, 0.000000000000000000, 1.000000000000000000 ) ) ;
#105425=FACE_BOUND ( 'NONE', #77473, .T. ) ;
#105426=ADVANCED_FACE ( 'NONE', ( #116041 ), #126330, .T. ) ;
#105427=CARTESIAN_POINT ( 'NONE',  ( 3.349999999999945466, 2.500000000000000000, -7.088010851410853519 ) ) ;
#105428=VECTOR ( 'NONE', #97323, 1000.000000000000000 ) ;
#105429=LINE ( 'NONE', #66772, #104970 ) ;
#105430=CARTESIAN_POINT ( 'NONE',  ( 12.89999999999989733, 2.500000000000000000, -0.1000000000000023925 ) ) ;
#105431=EDGE_CURVE ( 'NONE', #78527, #102277, #55227, .T. ) ;
#105432=ORIENTED_EDGE ( 'NONE', *, *, #4770, .T. ) ;
#105433=CARTESIAN_POINT ( 'NONE',  ( -12.04999999999999538, 2.500000000000000000, 6.595190528383296780 ) ) ;
#105434=DIRECTION ( 'NONE',  ( 0.000000000000000000, 1.000000000000000000, 0.000000000000000000 ) ) ;
#105435=ADVANCED_FACE ( 'NONE', ( #97685 ), #26386, .T. ) ;
#105436=CARTESIAN_POINT ( 'NONE',  ( 10.84999999999991260, 12.50000000000000000, 5.802370205355744659 ) ) ;
#105437=DIRECTION ( 'NONE',  ( 0.000000000000000000, 0.000000000000000000, 1.000000000000000000 ) ) ;
#105438=EDGE_LOOP ( 'NONE', ( #28115, #69741, #26909, #104892 ) ) ;
#105439=AXIS2_PLACEMENT_3D ( 'NONE', #86448, #99997, #99355 ) ;
#105440=CIRCLE ( 'NONE', #30245, 0.06509327318403745899 ) ;
#105441=DIRECTION ( 'NONE',  ( 0.000000000000000000, 1.000000000000000000, 0.000000000000000000 ) ) ;
#105442=EDGE_CURVE ( 'NONE', #30638, #32427, #68223, .T. ) ;
#105443=FACE_OUTER_BOUND ( 'NONE', #26463, .T. ) ;
#105444=ORIENTED_EDGE ( 'NONE', *, *, #96280, .F. ) ;
#105445=CARTESIAN_POINT ( 'NONE',  ( 3.549999999999942979, 12.50000000000000000, 1.818653347947321475 ) ) ;
#105446=EDGE_CURVE ( 'NONE', #126915, #44564, #65649, .T. ) ;
#105447=ORIENTED_EDGE ( 'NONE', *, *, #13986, .F. ) ;
#105448=FACE_BOUND ( 'NONE', #11438, .T. ) ;
#105449=EDGE_CURVE ( 'NONE', #84838, #58093, #36462, .T. ) ;
#105450=CARTESIAN_POINT ( 'NONE',  ( 7.099999999999928590, 12.50000000000000000, 4.330127018922196314 ) ) ;
#105451=ORIENTED_EDGE ( 'NONE', *, *, #63914, .F. ) ;
#105452=CARTESIAN_POINT ( 'NONE',  ( 6.249999999999968914, 2.500000000000000000, -6.595190528383302109 ) ) ;
#105453=DIRECTION ( 'NONE',  ( 0.000000000000000000, 0.000000000000000000, -1.000000000000000000 ) ) ;
#105454=VERTEX_POINT ( 'NONE', #16530 ) ;
#105455=ORIENTED_EDGE ( 'NONE', *, *, #118446, .F. ) ;
#105457=EDGE_LOOP ( 'NONE', ( #91714, #89185 ) ) ;
#105459=DIRECTION ( 'NONE',  ( 0.000000000000000000, 1.000000000000000000, 0.000000000000000000 ) ) ;
#105461=CIRCLE ( 'NONE', #90881, 0.06509327318403745899 ) ;
#105462=CARTESIAN_POINT ( 'NONE',  ( 3.149999999999946176, 2.500000000000000000, -1.918653347947325782 ) ) ;
#105463=DIRECTION ( 'NONE',  ( 0.000000000000000000, -0.000000000000000000, 1.000000000000000000 ) ) ;
#105464=DIRECTION ( 'NONE',  ( 0.000000000000000000, 0.000000000000000000, 1.000000000000000000 ) ) ;
#105465=AXIS2_PLACEMENT_3D ( 'NONE', #29773, #69698, #109632 ) ;
#105466=ORIENTED_EDGE ( 'NONE', *, *, #122880, .F. ) ;
#105467=VERTEX_POINT ( 'NONE', #88503 ) ;
#105468=DIRECTION ( 'NONE',  ( 0.000000000000000000, 0.000000000000000000, 1.000000000000000000 ) ) ;
#105469=CARTESIAN_POINT ( 'NONE',  ( 10.19999999999991225, 2.500000000000000000, -4.776537180435978414 ) ) ;
#105470=DIRECTION ( 'NONE',  ( 0.000000000000000000, 0.000000000000000000, 1.000000000000000000 ) ) ;
#105471=DIRECTION ( 'NONE',  ( 0.000000000000000000, 0.000000000000000000, 1.000000000000000000 ) ) ;
#105472=ORIENTED_EDGE ( 'NONE', *, *, #60029, .F. ) ;
#105473=ORIENTED_EDGE ( 'NONE', *, *, #4436, .F. ) ;
#105474=FACE_BOUND ( 'NONE', #105410, .T. ) ;
#105476=DIRECTION ( 'NONE',  ( 0.000000000000000000, 0.000000000000000000, 1.000000000000000000 ) ) ;
#105477=FACE_OUTER_BOUND ( 'NONE', #29233, .T. ) ;
#105478=ORIENTED_EDGE ( 'NONE', *, *, #112943, .T. ) ;
#105479=CARTESIAN_POINT ( 'NONE',  ( 12.04999999999990834, 12.50000000000000000, 6.495190528383297135 ) ) ;
#105481=ADVANCED_FACE ( 'NONE', ( #66295 ), #75467, .T. ) ;
#105482=CARTESIAN_POINT ( 'NONE',  ( 8.549999999999920774, 12.50000000000000000, 6.083687093685483660 ) ) ;
#105483=VECTOR ( 'NONE', #94253, 1000.000000000000000 ) ;
#105484=DIRECTION ( 'NONE',  ( 0.000000000000000000, -0.000000000000000000, 1.000000000000000000 ) ) ;
#105485=AXIS2_PLACEMENT_3D ( 'NONE', #16797, #86852, #56722 ) ;
#105486=CARTESIAN_POINT ( 'NONE',  ( 7.899999999999924860, 2.500000000000000000, -5.022947341949754119 ) ) ;
#105487=ADVANCED_FACE ( 'NONE', ( #126515 ), #105397, .T. ) ;
#105488=CARTESIAN_POINT ( 'NONE',  ( -12.49999999999999467, 2.500000000000000000, 0.7928203230275536750 ) ) ;
#105489=AXIS2_PLACEMENT_3D ( 'NONE', #97796, #87319, #49369 ) ;
#105490=AXIS2_PLACEMENT_3D ( 'NONE', #77617, #59306, #27886 ) ;
#105491=CARTESIAN_POINT ( 'NONE',  ( 11.64999999999990443, 2.500000000000000000, 2.957883832488649389 ) ) ;
#105492=DIRECTION ( 'NONE',  ( -0.000000000000000000, -1.000000000000000000, -0.000000000000000000 ) ) ;
#105493=DIRECTION ( 'NONE',  ( -0.000000000000000000, 1.000000000000000000, -0.000000000000000000 ) ) ;
#105494=AXIS2_PLACEMENT_3D ( 'NONE', #94881, #45153, #35328 ) ;
#105495=ORIENTED_EDGE ( 'NONE', *, *, #94206, .T. ) ;
#105496=CONICAL_SURFACE ( 'NONE', #111749, 0.1000000000000000472, 0.003490658503988666988 ) ;
#105497=EDGE_LOOP ( 'NONE', ( #42576, #125849, #73666, #72532 ) ) ;
#105498=AXIS2_PLACEMENT_3D ( 'NONE', #20684, #32462, #21986 ) ;
#105499=DIRECTION ( 'NONE',  ( 0.000000000000000000, 0.000000000000000000, 1.000000000000000000 ) ) ;
#105500=ORIENTED_EDGE ( 'NONE', *, *, #57573, .T. ) ;
#105501=DIRECTION ( 'NONE',  ( -4.274815082592931898E-19, -0.9999939076577903929, -0.003490651415223739937 ) ) ;
#105502=VERTEX_POINT ( 'NONE', #19784 ) ;
#105503=VERTEX_POINT ( 'NONE', #82425 ) ;
#105504=ORIENTED_EDGE ( 'NONE', *, *, #4954, .T. ) ;
#105505=CARTESIAN_POINT ( 'NONE',  ( -2.900000000000030109, 12.50000000000000000, -3.702399969078687292 ) ) ;
#105506=AXIS2_PLACEMENT_3D ( 'NONE', #116940, #27280, #17450 ) ;
#105507=VECTOR ( 'NONE', #92920, 1000.000000000000000 ) ;
#105508=DIRECTION ( 'NONE',  ( 0.000000000000000000, 1.000000000000000000, 0.000000000000000000 ) ) ;
#105509=DIRECTION ( 'NONE',  ( 0.000000000000000000, 0.000000000000000000, 1.000000000000000000 ) ) ;
#105510=CARTESIAN_POINT ( 'NONE',  ( 7.899999999999924860, 12.50000000000000000, -4.330127018922201643 ) ) ;
#105511=AXIS2_PLACEMENT_3D ( 'NONE', #73180, #23421, #84279 ) ;
#105512=FACE_OUTER_BOUND ( 'NONE', #87278, .T. ) ;
#105513=ORIENTED_EDGE ( 'NONE', *, *, #32619, .T. ) ;
#105514=FACE_OUTER_BOUND ( 'NONE', #121726, .T. ) ;
#105515=VERTEX_POINT ( 'NONE', #79355 ) ;
#105516=ORIENTED_EDGE ( 'NONE', *, *, #646, .T. ) ;
#105517=VERTEX_POINT ( 'NONE', #32037 ) ;
#105518=ORIENTED_EDGE ( 'NONE', *, *, #109039, .F. ) ;
#105519=CARTESIAN_POINT ( 'NONE',  ( 10.84999999999990905, 2.500000000000000000, -6.595190528383302109 ) ) ;
#105520=ORIENTED_EDGE ( 'NONE', *, *, #118879, .F. ) ;
#105521=ORIENTED_EDGE ( 'NONE', *, *, #87473, .F. ) ;
#105522=AXIS2_PLACEMENT_3D ( 'NONE', #57401, #105201, #76400 ) ;
#105523=CARTESIAN_POINT ( 'NONE',  ( 5.849999999999935696, 2.500000000000000000, -7.188010851410854052 ) ) ;
#105524=EDGE_CURVE ( 'NONE', #25026, #129352, #48977, .T. ) ;
#105525=CARTESIAN_POINT ( 'NONE',  ( -2.500000000000032863, 12.50000000000000000, 5.088040615133786027 ) ) ;
#105526=DIRECTION ( 'NONE',  ( 0.000000000000000000, 0.000000000000000000, 1.000000000000000000 ) ) ;
#105527=CARTESIAN_POINT ( 'NONE',  ( 8.549999999999920774, 2.500000000000000000, 6.048780366869521252 ) ) ;
#105528=LINE ( 'NONE', #15842, #97256 ) ;
#105529=CARTESIAN_POINT ( 'NONE',  ( -5.600000000000023626, 12.50000000000000000, -4.676537180435977881 ) ) ;
#105530=ORIENTED_EDGE ( 'NONE', *, *, #59802, .F. ) ;
#105531=DIRECTION ( 'NONE',  ( 0.000000000000000000, 0.000000000000000000, 1.000000000000000000 ) ) ;
#105532=AXIS2_PLACEMENT_3D ( 'NONE', #36422, #84853, #55402 ) ;
#105533=EDGE_CURVE ( 'NONE', #80302, #7899, #39449, .T. ) ;
#105534=AXIS2_PLACEMENT_3D ( 'NONE', #20122, #60068, #22715 ) ;
#105535=ORIENTED_EDGE ( 'NONE', *, *, #77254, .F. ) ;
#105536=DIRECTION ( 'NONE',  ( 0.000000000000000000, 1.000000000000000000, 0.000000000000000000 ) ) ;
#105537=ORIENTED_EDGE ( 'NONE', *, *, #65626, .T. ) ;
#105538=CARTESIAN_POINT ( 'NONE',  ( -0.6500000000000389910, 2.500000000000000000, -6.148780366869526226 ) ) ;
#105539=EDGE_LOOP ( 'NONE', ( #123558, #9198 ) ) ;
#105540=EDGE_CURVE ( 'NONE', #60348, #87315, #42731, .T. ) ;
#105541=EDGE_CURVE ( 'NONE', #107815, #3627, #19724, .T. ) ;
#105542=ORIENTED_EDGE ( 'NONE', *, *, #103168, .T. ) ;
#105544=DIRECTION ( 'NONE',  ( 0.000000000000000000, -0.000000000000000000, 1.000000000000000000 ) ) ;
#105545=CARTESIAN_POINT ( 'NONE',  ( -2.500000000000032419, 12.50000000000000000, 0.6928203230275494784 ) ) ;
#105546=AXIS2_PLACEMENT_3D ( 'NONE', #125221, #116037, #65645 ) ;
#105548=DIRECTION ( 'NONE',  ( -0.000000000000000000, -1.000000000000000000, -0.000000000000000000 ) ) ;
#105549=DIRECTION ( 'NONE',  ( -0.000000000000000000, 1.000000000000000000, -0.000000000000000000 ) ) ;
#105550=ORIENTED_EDGE ( 'NONE', *, *, #54396, .T. ) ;
#105551=DIRECTION ( 'NONE',  ( 0.000000000000000000, 0.000000000000000000, 1.000000000000000000 ) ) ;
#105552=DIRECTION ( 'NONE',  ( 0.000000000000000000, -0.9999939076577903929, 0.003490651415223739937 ) ) ;
#105553=EDGE_CURVE ( 'NONE', #70010, #22461, #103352, .T. ) ;
#105554=LINE ( 'NONE', #127762, #60687 ) ;
#105555=DIRECTION ( 'NONE',  ( 0.000000000000000000, -0.000000000000000000, 1.000000000000000000 ) ) ;
#105556=DIRECTION ( 'NONE',  ( 0.000000000000000000, 0.000000000000000000, -1.000000000000000000 ) ) ;
#105557=VERTEX_POINT ( 'NONE', #9957 ) ;
#105558=AXIS2_PLACEMENT_3D ( 'NONE', #81761, #60847, #102065 ) ;
#105559=CIRCLE ( 'NONE', #13596, 0.1000000000000002554 ) ;
#105560=ORIENTED_EDGE ( 'NONE', *, *, #90543, .F. ) ;
#105561=UNCERTAINTY_MEASURE_WITH_UNIT (LENGTH_MEASURE( 1.000000000000000082E-05 ), #92451, 'distance_accuracy_value', 'NONE');
#105562=ORIENTED_EDGE ( 'NONE', *, *, #49179, .F. ) ;
#105563=CARTESIAN_POINT ( 'NONE',  ( -4.350000000000023626, 2.500000000000000000, -1.718653347947325827 ) ) ;
#105564=DIRECTION ( 'NONE',  ( 0.000000000000000000, 1.000000000000000000, 0.000000000000000000 ) ) ;
#105566=LINE ( 'NONE', #123272, #34413 ) ;
#105567=DIRECTION ( 'NONE',  ( 0.000000000000000000, 1.000000000000000000, 0.000000000000000000 ) ) ;
#105568=FACE_OUTER_BOUND ( 'NONE', #35021, .T. ) ;
#105569=AXIS2_PLACEMENT_3D ( 'NONE', #35331, #15003, #123677 ) ;
#105570=CARTESIAN_POINT ( 'NONE',  ( 12.09999999999990550, 12.50000000000000000, -4.395220292106239768 ) ) ;
#105571=VERTEX_POINT ( 'NONE', #49899 ) ;
#105572=EDGE_CURVE ( 'NONE', #55495, #66544, #3211, .T. ) ;
#105573=CIRCLE ( 'NONE', #88838, 0.1000000000000000472 ) ;
#105574=FACE_OUTER_BOUND ( 'NONE', #89116, .T. ) ;
#105575=DIRECTION ( 'NONE',  ( -0.000000000000000000, 1.000000000000000000, -0.000000000000000000 ) ) ;
#105576=CONICAL_SURFACE ( 'NONE', #5297, 0.09999999999999982514, 0.003490658503988666988 ) ;
#105577=ORIENTED_EDGE ( 'NONE', *, *, #92669, .F. ) ;
#105578=AXIS2_PLACEMENT_3D ( 'NONE', #28225, #29512, #79891 ) ;
#105579=EDGE_CURVE ( 'NONE', #110110, #20105, #103342, .T. ) ;
#105580=DIRECTION ( 'NONE',  ( -4.274815082592931898E-19, -0.9999939076577903929, -0.003490651415223739937 ) ) ;
#105581=DIRECTION ( 'NONE',  ( 0.000000000000000000, 0.000000000000000000, 1.000000000000000000 ) ) ;
#105582=EDGE_CURVE ( 'NONE', #54150, #70834, #97075, .T. ) ;
#105583=DIRECTION ( 'NONE',  ( 0.000000000000000000, -0.9999939076577903929, 0.003490651415223739937 ) ) ;
#105584=AXIS2_PLACEMENT_3D ( 'NONE', #46935, #94719, #37745 ) ;
#105585=AXIS2_PLACEMENT_3D ( 'NONE', #105323, #104035, #94857 ) ;
#105586=EDGE_LOOP ( 'NONE', ( #91911, #99890 ) ) ;
#105587=AXIS2_PLACEMENT_3D ( 'NONE', #72848, #70917, #11983 ) ;
#105588=DIRECTION ( 'NONE',  ( -0.000000000000000000, -1.000000000000000000, -0.000000000000000000 ) ) ;
#105589=ADVANCED_FACE ( 'NONE', ( #33324 ), #12667, .T. ) ;
#105590=CONICAL_SURFACE ( 'NONE', #49174, 0.09999999999999982514, 0.003490658503988666988 ) ;
#105591=EDGE_CURVE ( 'NONE', #56070, #4982, #41950, .T. ) ;
#105592=ORIENTED_EDGE ( 'NONE', *, *, #118436, .T. ) ;
#105593=CARTESIAN_POINT ( 'NONE',  ( 1.849999999999949019, 2.500000000000000000, 6.941600689897073018 ) ) ;
#105594=FACE_OUTER_BOUND ( 'NONE', #29106, .T. ) ;
#105595=EDGE_CURVE ( 'NONE', #33970, #28402, #94161, .T. ) ;
#105596=EDGE_CURVE ( 'NONE', #90021, #124886, #110871, .T. ) ;
#105597=ORIENTED_EDGE ( 'NONE', *, *, #42349, .T. ) ;
#105598=CONICAL_SURFACE ( 'NONE', #78515, 0.1000000000000002554, 0.003490658503988666988 ) ;
#105599=VECTOR ( 'NONE', #12087, 1000.000000000000000 ) ;
#105600=DIRECTION ( 'NONE',  ( -0.000000000000000000, -1.000000000000000000, -0.000000000000000000 ) ) ;
#105601=EDGE_CURVE ( 'NONE', #36661, #55739, #35682, .T. ) ;
#105602=PLANE ( 'NONE',  #108122 ) ;
#105603=VECTOR ( 'NONE', #22013, 1000.000000000000000 ) ;
#105604=VERTEX_POINT ( 'NONE', #62776 ) ;
#105605=EDGE_CURVE ( 'NONE', #79633, #94125, #71952, .T. ) ;
#105606=FACE_OUTER_BOUND ( 'NONE', #115738, .T. ) ;
#105607=EDGE_LOOP ( 'NONE', ( #48196, #114214, #75703, #112749 ) ) ;
#105608=VERTEX_POINT ( 'NONE', #92209 ) ;
#105609=CARTESIAN_POINT ( 'NONE',  ( 3.349999999999942801, 2.500000000000000000, 2.957883832488649389 ) ) ;
#105610=CARTESIAN_POINT ( 'NONE',  ( -6.850000000000013856, 2.500000000000000000, 1.918653347947321564 ) ) ;
#105611=EDGE_LOOP ( 'NONE', ( #22177, #24826, #116408, #93898 ) ) ;
#105612=CARTESIAN_POINT ( 'NONE',  ( 2.699999999999946443, 12.50000000000000000, 0.4115034346978109769 ) ) ;
#105613=PLANE ( 'NONE',  #98620 ) ;
#105614=CIRCLE ( 'NONE', #90942, 0.06509327318403745899 ) ;
#105615=ORIENTED_EDGE ( 'NONE', *, *, #30894, .T. ) ;
#105616=LINE ( 'NONE', #94481, #9169 ) ;
#105617=DIRECTION ( 'NONE',  ( 0.000000000000000000, 0.000000000000000000, 1.000000000000000000 ) ) ;
#105618=CARTESIAN_POINT ( 'NONE',  ( 17.02136413300351947, -1.939324994459653118, -5.540650668389590194 ) ) ;
#105619=DIRECTION ( 'NONE',  ( -4.274815082592931898E-19, -0.9999939076577903929, -0.003490651415223739937 ) ) ;
#105620=CARTESIAN_POINT ( 'NONE',  ( 14.39999999999989555, 12.50000000000000000, 0.3464101615137736845 ) ) ;
#105621=CIRCLE ( 'NONE', #22015, 0.1000000000000002554 ) ;
#105622=CARTESIAN_POINT ( 'NONE',  ( -13.34999999999999076, 2.500000000000000000, 1.472243186433549456 ) ) ;
#105623=AXIS2_PLACEMENT_3D ( 'NONE', #92596, #72326, #91952 ) ;
#105624=AXIS2_PLACEMENT_3D ( 'NONE', #16072, #124763, #126038 ) ;
#105625=VERTEX_POINT ( 'NONE', #2533 ) ;
#105627=VERTEX_POINT ( 'NONE', #42496 ) ;
#105628=EDGE_LOOP ( 'NONE', ( #36449, #86379 ) ) ;
#105629=LINE ( 'NONE', #103035, #28603 ) ;
#105630=DIRECTION ( 'NONE',  ( 0.000000000000000000, 1.000000000000000000, 0.000000000000000000 ) ) ;
#105631=DIRECTION ( 'NONE',  ( -0.000000000000000000, 1.000000000000000000, -0.000000000000000000 ) ) ;
#105632=ORIENTED_EDGE ( 'NONE', *, *, #46976, .F. ) ;
#105633=FACE_BOUND ( 'NONE', #42219, .T. ) ;
#105634=FACE_OUTER_BOUND ( 'NONE', #20653, .T. ) ;
#105635=CARTESIAN_POINT ( 'NONE',  ( -12.04999999999999716, 12.50000000000000000, -2.165063509461097713 ) ) ;
#105636=CIRCLE ( 'NONE', #7322, 0.09999999999999982514 ) ;
#105637=DIRECTION ( 'NONE',  ( 0.000000000000000000, 1.000000000000000000, 0.000000000000000000 ) ) ;
#105638=EDGE_CURVE ( 'NONE', #10224, #97917, #54446, .T. ) ;
#105639=LINE ( 'NONE', #6127, #63797 ) ;
#105640=AXIS2_PLACEMENT_3D ( 'NONE', #41739, #111746, #122219 ) ;
#105641=LINE ( 'NONE', #15941, #63893 ) ;
#105642=CARTESIAN_POINT ( 'NONE',  ( 2.099999999999948574, 2.500000000000000000, 4.430127018922196847 ) ) ;
#105643=CARTESIAN_POINT ( 'NONE',  ( -4.150000000000025224, 2.500000000000000000, 2.757883832488649656 ) ) ;
#105644=DIRECTION ( 'NONE',  ( 0.000000000000000000, 1.000000000000000000, 0.000000000000000000 ) ) ;
#105645=DIRECTION ( 'NONE',  ( 0.000000000000000000, 0.000000000000000000, -1.000000000000000000 ) ) ;
#105646=FACE_OUTER_BOUND ( 'NONE', #38480, .T. ) ;
#105647=ADVANCED_FACE ( 'NONE', ( #52952 ), #56496, .T. ) ;
#105648=VECTOR ( 'NONE', #57961, 1000.000000000000000 ) ;
#105649=VERTEX_POINT ( 'NONE', #19102 ) ;
#105651=ORIENTED_EDGE ( 'NONE', *, *, #114143, .F. ) ;
#105652=EDGE_LOOP ( 'NONE', ( #20774, #70876, #110662, #104728 ) ) ;
#105653=CARTESIAN_POINT ( 'NONE',  ( 2.899999999999945732, 12.50000000000000000, -2.385244779468109755E-15 ) ) ;
#105654=EDGE_LOOP ( 'NONE', ( #17586, #49807 ) ) ;
#105655=PLANE ( 'NONE',  #109132 ) ;
#105656=VERTEX_POINT ( 'NONE', #59061 ) ;
#105657=EDGE_LOOP ( 'NONE', ( #61189, #99098, #50241, #14672 ) ) ;
#105658=CARTESIAN_POINT ( 'NONE',  ( -1.900000000000034994, 12.50000000000000000, -0.3464101615137783474 ) ) ;
#105659=AXIS2_PLACEMENT_3D ( 'NONE', #91480, #81659, #100023 ) ;
#105661=CARTESIAN_POINT ( 'NONE',  ( -13.54999999999999005, 2.500000000000000000, -1.818653347947323917 ) ) ;
#105662=PLANE ( 'NONE',  #20682 ) ;
#105664=FACE_OUTER_BOUND ( 'NONE', #94115, .T. ) ;
#105666=EDGE_LOOP ( 'NONE', ( #83243, #9488, #17376, #34291 ) ) ;
#105667=ORIENTED_EDGE ( 'NONE', *, *, #101864, .F. ) ;
#105668=CONICAL_SURFACE ( 'NONE', #101460, 0.09999999999999999167, 0.003490658503988666988 ) ;
#105669=VERTEX_POINT ( 'NONE', #64053 ) ;
#105670=ORIENTED_EDGE ( 'NONE', *, *, #54792, .T. ) ;
#105672=CARTESIAN_POINT ( 'NONE',  ( -9.600000000000006750, 12.50000000000000000, -0.6928203230275542523 ) ) ;
#105673=EDGE_LOOP ( 'NONE', ( #419, #103722 ) ) ;
#105674=VERTEX_POINT ( 'NONE', #24779 ) ;
#105675=FACE_OUTER_BOUND ( 'NONE', #48329, .T. ) ;
#105676=CIRCLE ( 'NONE', #65953, 0.1000000000000000056 ) ;
#105677=ADVANCED_FACE ( 'NONE', ( #65980 ), #64906, .T. ) ;
#105678=CARTESIAN_POINT ( 'NONE',  ( -4.800000000000028244, 12.50000000000000000, -3.983716857408426293 ) ) ;
#105679=DIRECTION ( 'NONE',  ( 0.000000000000000000, 1.000000000000000000, 0.000000000000000000 ) ) ;
#105680=CARTESIAN_POINT ( 'NONE',  ( 7.699999999999925571, 12.50000000000000000, 4.048810130592458201 ) ) ;
#105681=AXIS2_PLACEMENT_3D ( 'NONE', #37643, #25873, #5567 ) ;
#105682=DIRECTION ( 'NONE',  ( 0.000000000000000000, 0.000000000000000000, -1.000000000000000000 ) ) ;
#105684=EDGE_LOOP ( 'NONE', ( #34085, #28968 ) ) ;
#105685=CARTESIAN_POINT ( 'NONE',  ( -2.300000000000033129, 12.50000000000000000, 3.918623584224382839 ) ) ;
#105686=CIRCLE ( 'NONE', #3277, 0.06509327318403745899 ) ;
#105687=VECTOR ( 'NONE', #98370, 1000.000000000000000 ) ;
#105688=EDGE_CURVE ( 'NONE', #87698, #45516, #66, .T. ) ;
#105689=ORIENTED_EDGE ( 'NONE', *, *, #27423, .T. ) ;
#105690=DIRECTION ( 'NONE',  ( -0.000000000000000000, -1.000000000000000000, -0.000000000000000000 ) ) ;
#105691=VECTOR ( 'NONE', #32281, 1000.000000000000000 ) ;
#105692=EDGE_LOOP ( 'NONE', ( #106008, #72070 ) ) ;
#105693=CARTESIAN_POINT ( 'NONE',  ( -2.950000000000029932, 2.500000000000000000, -2.165063509461101710 ) ) ;
#105694=FACE_OUTER_BOUND ( 'NONE', #19451, .T. ) ;
#105695=AXIS2_PLACEMENT_3D ( 'NONE', #110058, #111313, #21679 ) ;
#105696=EDGE_LOOP ( 'NONE', ( #128634, #74854 ) ) ;
#105697=DIRECTION ( 'NONE',  ( -0.000000000000000000, -1.000000000000000000, -0.000000000000000000 ) ) ;
#105698=ADVANCED_FACE ( 'NONE', ( #103983 ), #125548, .T. ) ;
#105699=DIRECTION ( 'NONE',  ( 0.000000000000000000, 1.000000000000000000, 0.000000000000000000 ) ) ;
#105700=EDGE_CURVE ( 'NONE', #118817, #34687, #121343, .T. ) ;
#105701=ORIENTED_EDGE ( 'NONE', *, *, #32031, .T. ) ;
#105702=CARTESIAN_POINT ( 'NONE',  ( -14.39999999999998614, 2.500000000000000000, -0.2464101615137760659 ) ) ;
#105703=EDGE_CURVE ( 'NONE', #85431, #121481, #6381, .T. ) ;
#105704=CARTESIAN_POINT ( 'NONE',  ( 10.59999999999991260, 12.50000000000000000, -0.3464101615137783474 ) ) ;
#105705=ORIENTED_EDGE ( 'NONE', *, *, #3200, .F. ) ;
#105707=CARTESIAN_POINT ( 'NONE',  ( -11.64999999999999680, 12.50000000000000000, -7.122917578226813262 ) ) ;
#105708=CARTESIAN_POINT ( 'NONE',  ( 11.89999999999990798, 2.500000000000000000, -4.083716857408426826 ) ) ;
#105709=EDGE_CURVE ( 'NONE', #81765, #35406, #102483, .T. ) ;
#105711=AXIS2_PLACEMENT_3D ( 'NONE', #106741, #38013, #75999 ) ;
#105712=CARTESIAN_POINT ( 'NONE',  ( -8.150000000000012790, 2.500000000000000000, 2.511473670974873507 ) ) ;
#105713=CARTESIAN_POINT ( 'NONE',  ( 0.4499999999999573785, 2.500000000000000000, -6.495190528383302464 ) ) ;
#105714=FACE_OUTER_BOUND ( 'NONE', #106412, .T. ) ;
#105715=CIRCLE ( 'NONE', #107851, 0.1000000000000000056 ) ;
#105716=AXIS2_PLACEMENT_3D ( 'NONE', #44108, #64393, #73556 ) ;
#105717=ORIENTED_EDGE ( 'NONE', *, *, #104692, .T. ) ;
#105718=CIRCLE ( 'NONE', #40985, 0.1000000000000002554 ) ;
#105719=CARTESIAN_POINT ( 'NONE',  ( 15.79999999999989058, 2.500000000000000000, -0.1000000000000023925 ) ) ;
#105720=VERTEX_POINT ( 'NONE', #14291 ) ;
#105721=DIRECTION ( 'NONE',  ( -0.000000000000000000, 1.000000000000000000, -0.000000000000000000 ) ) ;
#105722=DIRECTION ( 'NONE',  ( 0.000000000000000000, 0.000000000000000000, 1.000000000000000000 ) ) ;
#105723=DIRECTION ( 'NONE',  ( -0.000000000000000000, 1.000000000000000000, -0.000000000000000000 ) ) ;
#105724=VERTEX_POINT ( 'NONE', #114429 ) ;
#105725=AXIS2_PLACEMENT_3D ( 'NONE', #89654, #98813, #99483 ) ;
#105726=VECTOR ( 'NONE', #60896, 1000.000000000000000 ) ;
#105727=CIRCLE ( 'NONE', #55643, 0.1000000000000000472 ) ;
#105728=LINE ( 'NONE', #116173, #26360 ) ;
#105729=PLANE ( 'NONE',  #1597 ) ;
#105730=ORIENTED_EDGE ( 'NONE', *, *, #93143, .T. ) ;
#105731=DIRECTION ( 'NONE',  ( -0.000000000000000000, -1.000000000000000000, -0.000000000000000000 ) ) ;
#105732=CONICAL_SURFACE ( 'NONE', #93135, 0.1000000000000002554, 0.003490658503988666988 ) ;
#105733=EDGE_LOOP ( 'NONE', ( #98064, #23502, #8592, #51346 ) ) ;
#105734=ORIENTED_EDGE ( 'NONE', *, *, #48875, .T. ) ;
#105735=DIRECTION ( 'NONE',  ( 0.000000000000000000, 0.000000000000000000, -1.000000000000000000 ) ) ;
#105736=EDGE_CURVE ( 'NONE', #28294, #27245, #85619, .T. ) ;
#105737=ADVANCED_FACE ( 'NONE', ( #93515 ), #86249, .T. ) ;
#105738=VERTEX_POINT ( 'NONE', #4449 ) ;
#105739=DIRECTION ( 'NONE',  ( 0.000000000000000000, -0.000000000000000000, 1.000000000000000000 ) ) ;
#105741=ADVANCED_FACE ( 'NONE', ( #105261 ), #37736, .T. ) ;
#105742=EDGE_CURVE ( 'NONE', #98508, #34124, #104610, .T. ) ;
#105743=CARTESIAN_POINT ( 'NONE',  ( 12.09999999999990195, 2.500000000000000000, 0.6928203230275494784 ) ) ;
#105744=VERTEX_POINT ( 'NONE', #115718 ) ;
#105745=FACE_BOUND ( 'NONE', #24436, .T. ) ;
#105746=EDGE_CURVE ( 'NONE', #110810, #33973, #8465, .T. ) ;
#105747=DIRECTION ( 'NONE',  ( 0.000000000000000000, 0.000000000000000000, -1.000000000000000000 ) ) ;
#105748=ORIENTED_EDGE ( 'NONE', *, *, #75664, .F. ) ;
#105749=DIRECTION ( 'NONE',  ( 0.000000000000000000, 1.000000000000000000, 0.000000000000000000 ) ) ;
#105751=ORIENTED_EDGE ( 'NONE', *, *, #118973, .T. ) ;
#105752=EDGE_CURVE ( 'NONE', #23200, #32927, #46056, .T. ) ;
#105753=ADVANCED_FACE ( 'NONE', ( #115062 ), #89950, .T. ) ;
#105754=CIRCLE ( 'NONE', #49347, 0.1000000000000000056 ) ;
#105755=ORIENTED_EDGE ( 'NONE', *, *, #77619, .T. ) ;
#105756=AXIS2_PLACEMENT_3D ( 'NONE', #118576, #108117, #17124 ) ;
#105757=ORIENTED_EDGE ( 'NONE', *, *, #18375, .F. ) ;
#105758=DIRECTION ( 'NONE',  ( 0.000000000000000000, -0.9999939076577903929, 0.003490651415223739937 ) ) ;
#105759=CARTESIAN_POINT ( 'NONE',  ( 6.714630671518470706, 1.500000000000127010, 9.763603585529398998 ) ) ;
#105760=DIRECTION ( 'NONE',  ( 0.000000000000000000, 0.000000000000000000, 1.000000000000000000 ) ) ;
#105761=FACE_BOUND ( 'NONE', #27513, .T. ) ;
#105762=ORIENTED_EDGE ( 'NONE', *, *, #93664, .F. ) ;
#105764=EDGE_CURVE ( 'NONE', #31868, #32290, #4255, .T. ) ;
#105765=CARTESIAN_POINT ( 'NONE',  ( 10.64999999999991331, 12.50000000000000000, 6.841600689897072485 ) ) ;
#105766=CARTESIAN_POINT ( 'NONE',  ( -6.900000000000019007, 2.500000000000000000, -3.983716857408426293 ) ) ;
#105767=CARTESIAN_POINT ( 'NONE',  ( -4.600000000000024514, 2.500000000000000000, -0.6928203230275542523 ) ) ;
#105768=DIRECTION ( 'NONE',  ( 0.000000000000000000, 0.000000000000000000, -1.000000000000000000 ) ) ;
#105770=CARTESIAN_POINT ( 'NONE',  ( 11.04999999999991012, 12.50000000000000000, 6.906693963081109722 ) ) ;
#105771=DIRECTION ( 'NONE',  ( -0.000000000000000000, 1.000000000000000000, -0.000000000000000000 ) ) ;
#105772=CONICAL_SURFACE ( 'NONE', #49262, 0.09999999999999999167, 0.003490658503988666988 ) ;
#105773=CARTESIAN_POINT ( 'NONE',  ( -2.950000000000029932, 2.500000000000000000, 2.165063509461097713 ) ) ;
#105774=AXIS2_PLACEMENT_3D ( 'NONE', #110651, #21636, #79906 ) ;
#105775=ORIENTED_EDGE ( 'NONE', *, *, #40138, .T. ) ;
#105776=VERTEX_POINT ( 'NONE', #94801 ) ;
#105777=EDGE_LOOP ( 'NONE', ( #46205, #81834 ) ) ;
#105778=VERTEX_POINT ( 'NONE', #76452 ) ;
#105779=CIRCLE ( 'NONE', #128787, 0.1000000000000002554 ) ;
#105780=ORIENTED_EDGE ( 'NONE', *, *, #79570, .T. ) ;
#105782=DIRECTION ( 'NONE',  ( -4.274815082592931898E-19, -0.9999939076577903929, -0.003490651415223739937 ) ) ;
#105783=EDGE_LOOP ( 'NONE', ( #15519, #102228 ) ) ;
#105784=FACE_BOUND ( 'NONE', #50304, .T. ) ;
#105785=CARTESIAN_POINT ( 'NONE',  ( -5.200000000000020606, 12.50000000000000000, -0.3464101615137782364 ) ) ;
#105786=DIRECTION ( 'NONE',  ( -0.000000000000000000, -1.000000000000000000, -0.000000000000000000 ) ) ;
#105787=CARTESIAN_POINT ( 'NONE',  ( 2.099999999999948574, 12.50000000000000000, 3.637306695894644726 ) ) ;
#105788=CARTESIAN_POINT ( 'NONE',  ( 13.29999999999990301, 2.500000000000000000, 4.330127018922196314 ) ) ;
#105789=CARTESIAN_POINT ( 'NONE',  ( 1.899999999999951283, 12.50000000000000000, -4.048810130592463530 ) ) ;
#105790=CONICAL_SURFACE ( 'NONE', #20028, 0.1000000000000002554, 0.003490658503988666988 ) ;
#105791=ORIENTED_EDGE ( 'NONE', *, *, #104336, .T. ) ;
#105792=DIRECTION ( 'NONE',  ( 0.000000000000000000, 0.000000000000000000, -1.000000000000000000 ) ) ;
#105793=VERTEX_POINT ( 'NONE', #116362 ) ;
#105794=EDGE_CURVE ( 'NONE', #9476, #3359, #117125, .T. ) ;
#105797=ORIENTED_EDGE ( 'NONE', *, *, #112779, .T. ) ;
#105798=CARTESIAN_POINT ( 'NONE',  ( 3.149999999999944400, 12.50000000000000000, 1.818653347947321475 ) ) ;
#105799=DIRECTION ( 'NONE',  ( 0.000000000000000000, 0.000000000000000000, 1.000000000000000000 ) ) ;
#105800=VECTOR ( 'NONE', #24182, 1000.000000000000000 ) ;
#105801=CARTESIAN_POINT ( 'NONE',  ( 4.549999999999939426, 2.500000000000000000, -6.495190528383302464 ) ) ;
#105802=EDGE_LOOP ( 'NONE', ( #21973, #13891, #41814, #82571 ) ) ;
#105803=CARTESIAN_POINT ( 'NONE',  ( 15.50772381900151942, 2.499999999999936939, -6.996973298636524952 ) ) ;
#105804=CIRCLE ( 'NONE', #114115, 0.06509327318403745899 ) ;
#105805=CONICAL_SURFACE ( 'NONE', #89167, 0.1000000000000002554, 0.003490658503988666988 ) ;
#105806=DIRECTION ( 'NONE',  ( 0.000000000000000000, 0.000000000000000000, 1.000000000000000000 ) ) ;
#105807=AXIS2_PLACEMENT_3D ( 'NONE', #97549, #18345, #117166 ) ;
#105808=DIRECTION ( 'NONE',  ( -0.000000000000000000, -1.000000000000000000, -0.000000000000000000 ) ) ;
#105810=CARTESIAN_POINT ( 'NONE',  ( -9.600000000000008527, 2.500000000000000000, -4.430127018922197735 ) ) ;
#105811=CARTESIAN_POINT ( 'NONE',  ( -1.650000000000034772, 12.50000000000000000, 1.537336459617582918 ) ) ;
#105812=ORIENTED_EDGE ( 'NONE', *, *, #34660, .T. ) ;
#105813=DIRECTION ( 'NONE',  ( -0.000000000000000000, -1.000000000000000000, -0.000000000000000000 ) ) ;
#105814=CIRCLE ( 'NONE', #11718, 0.09999999999999999167 ) ;
#105815=ORIENTED_EDGE ( 'NONE', *, *, #64874, .F. ) ;
#105816=AXIS2_PLACEMENT_3D ( 'NONE', #21464, #41775, #101325 ) ;
#105817=CIRCLE ( 'NONE', #66096, 0.09999999999999982514 ) ;
#105818=ORIENTED_EDGE ( 'NONE', *, *, #14386, .F. ) ;
#105819=DIRECTION ( 'NONE',  ( -0.000000000000000000, 1.000000000000000000, -0.000000000000000000 ) ) ;
#105820=DIRECTION ( 'NONE',  ( 0.000000000000000000, 1.000000000000000000, 0.000000000000000000 ) ) ;
#105821=DIRECTION ( 'NONE',  ( 0.000000000000000000, -0.000000000000000000, 1.000000000000000000 ) ) ;
#105822=EDGE_LOOP ( 'NONE', ( #23281, #36451, #20662, #26930 ) ) ;
#105824=CARTESIAN_POINT ( 'NONE',  ( 7.899999999999924860, 12.50000000000000000, -3.702399969078687292 ) ) ;
#105825=DIRECTION ( 'NONE',  ( -0.000000000000000000, 1.000000000000000000, -0.000000000000000000 ) ) ;
#105826=CARTESIAN_POINT ( 'NONE',  ( -11.25000000000000000, 2.500000000000000000, 2.857883832488649301 ) ) ;
#105827=VERTEX_POINT ( 'NONE', #65323 ) ;
#105828=ORIENTED_EDGE ( 'NONE', *, *, #120648, .F. ) ;
#105829=CARTESIAN_POINT ( 'NONE',  ( -7.700000000000014388, 12.50000000000000000, -4.676537180435977881 ) ) ;
#105830=ORIENTED_EDGE ( 'NONE', *, *, #120957, .F. ) ;
#105831=DIRECTION ( 'NONE',  ( -0.000000000000000000, -1.000000000000000000, -0.000000000000000000 ) ) ;
#105832=EDGE_CURVE ( 'NONE', #57299, #44421, #15578, .T. ) ;
#105833=LINE ( 'NONE', #16139, #42914 ) ;
#105834=ORIENTED_EDGE ( 'NONE', *, *, #120009, .T. ) ;
#105835=DIRECTION ( 'NONE',  ( 0.000000000000000000, 1.000000000000000000, 0.000000000000000000 ) ) ;
#105836=CARTESIAN_POINT ( 'NONE',  ( -6.450000000000014388, 12.50000000000000000, 1.818653347947321475 ) ) ;
#105837=DIRECTION ( 'NONE',  ( -0.000000000000000000, -1.000000000000000000, -0.000000000000000000 ) ) ;
#105838=ADVANCED_FACE ( 'NONE', ( #48281 ), #85744, .T. ) ;
#105839=CARTESIAN_POINT ( 'NONE',  ( -0.6000000000000323963, 2.500000000000000000, -0.3464101615137759604 ) ) ;
#105840=EDGE_CURVE ( 'NONE', #105656, #63009, #119208, .T. ) ;
#105841=VERTEX_POINT ( 'NONE', #39772 ) ;
#105842=CARTESIAN_POINT ( 'NONE',  ( -14.14999999999998614, 2.500000000000000000, -2.165063509461099489 ) ) ;
#105843=AXIS2_PLACEMENT_3D ( 'NONE', #111421, #40793, #122560 ) ;
#105844=AXIS2_PLACEMENT_3D ( 'NONE', #120375, #71258, #39894 ) ;
#105845=DIRECTION ( 'NONE',  ( 0.000000000000000000, 0.000000000000000000, 1.000000000000000000 ) ) ;
#105846=EDGE_CURVE ( 'NONE', #51555, #54758, #104619, .T. ) ;
#105847=ORIENTED_EDGE ( 'NONE', *, *, #38316, .T. ) ;
#105848=EDGE_CURVE ( 'NONE', #128976, #54553, #6307, .T. ) ;
#105849=ORIENTED_EDGE ( 'NONE', *, *, #109057, .T. ) ;
#105850=ADVANCED_FACE ( 'NONE', ( #27993 ), #96202, .T. ) ;
#105852=CARTESIAN_POINT ( 'NONE',  ( 5.399999999999935518, 2.500000000000000000, -4.330127018922201643 ) ) ;
#105853=ADVANCED_FACE ( 'NONE', ( #29936 ), #27326, .T. ) ;
#105854=DIRECTION ( 'NONE',  ( 0.000000000000000000, 0.000000000000000000, -1.000000000000000000 ) ) ;
#105855=ADVANCED_FACE ( 'NONE', ( #97374 ), #117633, .T. ) ;
#105857=FACE_OUTER_BOUND ( 'NONE', #51632, .T. ) ;
#105858=DIRECTION ( 'NONE',  ( -0.000000000000000000, 1.000000000000000000, -0.000000000000000000 ) ) ;
#105859=CONICAL_SURFACE ( 'NONE', #99606, 0.1000000000000000472, 0.003490658503988666988 ) ;
#105860=CARTESIAN_POINT ( 'NONE',  ( 5.599999999999933031, 12.50000000000000000, -0.3464101615137783474 ) ) ;
#105861=CARTESIAN_POINT ( 'NONE',  ( 13.94999999999989271, 12.50000000000000000, -1.818653347947326138 ) ) ;
#105862=CARTESIAN_POINT ( 'NONE',  ( 11.04999999999991189, 12.50000000000000000, -2.511473670974877948 ) ) ;
#105863=EDGE_CURVE ( 'NONE', #25898, #57277, #16771, .T. ) ;
#105864=CARTESIAN_POINT ( 'NONE',  ( -6.450000000000017941, 2.500000000000000000, -6.941600689897077459 ) ) ;
#105865=AXIS2_PLACEMENT_3D ( 'NONE', #2833, #44699, #95084 ) ;
#105866=AXIS2_PLACEMENT_3D ( 'NONE', #119922, #32849, #23014 ) ;
#105867=ORIENTED_EDGE ( 'NONE', *, *, #45030, .T. ) ;
#105868=AXIS2_PLACEMENT_3D ( 'NONE', #107920, #115132, #47086 ) ;
#105869=ORIENTED_EDGE ( 'NONE', *, *, #3279, .T. ) ;
#105870=DIRECTION ( 'NONE',  ( 0.000000000000000000, 0.000000000000000000, -1.000000000000000000 ) ) ;
#105871=ORIENTED_EDGE ( 'NONE', *, *, #113412, .F. ) ;
#105872=CARTESIAN_POINT ( 'NONE',  ( -13.34999999999999076, 12.50000000000000000, -1.472243186433547901 ) ) ;
#105873=DIRECTION ( 'NONE',  ( 0.000000000000000000, 0.000000000000000000, 1.000000000000000000 ) ) ;
#105874=LINE ( 'NONE', #113271, #35356 ) ;
#105875=ORIENTED_EDGE ( 'NONE', *, *, #73031, .T. ) ;
#105876=CARTESIAN_POINT ( 'NONE',  ( 8.749999999999921840, 2.500000000000000000, -5.802370205355749988 ) ) ;
#105877=LINE ( 'NONE', #77688, #17741 ) ;
#105878=CARTESIAN_POINT ( 'NONE',  ( -13.94999999999998863, 2.500000000000000000, 2.411473670974877415 ) ) ;
#105879=ORIENTED_EDGE ( 'NONE', *, *, #99843, .T. ) ;
#105880=CIRCLE ( 'NONE', #41066, 0.06509327318403745899 ) ;
#105881=DIRECTION ( 'NONE',  ( 0.000000000000000000, -0.9999939076577903929, 0.003490651415223739937 ) ) ;
#105882=VERTEX_POINT ( 'NONE', #99319 ) ;
#105883=AXIS2_PLACEMENT_3D ( 'NONE', #82082, #40901, #32376 ) ;
#105884=EDGE_LOOP ( 'NONE', ( #31287, #39733 ) ) ;
#105885=ORIENTED_EDGE ( 'NONE', *, *, #117922, .F. ) ;
#105886=ORIENTED_EDGE ( 'NONE', *, *, #13351, .F. ) ;
#105887=CARTESIAN_POINT ( 'NONE',  ( 12.89999999999989910, 12.50000000000000000, -0.7579135962115917113 ) ) ;
#105888=VECTOR ( 'NONE', #70541, 1000.000000000000000 ) ;
#105889=ADVANCED_FACE ( 'NONE', ( #69857 ), #16855, .T. ) ;
#105890=CONICAL_SURFACE ( 'NONE', #112159, 0.1000000000000002554, 0.003490658503988666988 ) ;
#105891=CARTESIAN_POINT ( 'NONE',  ( -1.650000000000035216, 2.500000000000000000, -5.802370205355749988 ) ) ;
#105892=DIRECTION ( 'NONE',  ( 0.000000000000000000, 1.000000000000000000, 0.000000000000000000 ) ) ;
#105893=EDGE_CURVE ( 'NONE', #59034, #107306, #73315, .T. ) ;
#105894=CONICAL_SURFACE ( 'NONE', #70393, 0.1000000000000002554, 0.003490658503988666988 ) ;
#105895=DIRECTION ( 'NONE',  ( 0.000000000000000000, 1.000000000000000000, 0.000000000000000000 ) ) ;
#105896=ORIENTED_EDGE ( 'NONE', *, *, #123033, .T. ) ;
#105897=AXIS2_PLACEMENT_3D ( 'NONE', #76104, #47942, #116020 ) ;
#105898=EDGE_CURVE ( 'NONE', #42353, #28403, #27335, .T. ) ;
#105899=DIRECTION ( 'NONE',  ( -0.000000000000000000, -1.000000000000000000, -0.000000000000000000 ) ) ;
#105900=ORIENTED_EDGE ( 'NONE', *, *, #56890, .T. ) ;
#105901=CARTESIAN_POINT ( 'NONE',  ( 43.31961220472146579, -2.029667686315419939, -5.113275312223934499 ) ) ;
#105902=LINE ( 'NONE', #7029, #7866 ) ;
#105903=CARTESIAN_POINT ( 'NONE',  ( 9.399999999999915090, 2.500000000000000000, -3.983716857408426293 ) ) ;
#105904=CARTESIAN_POINT ( 'NONE',  ( 18.93069778776427370, -2.571126379696592856, 2.451182541063249953 ) ) ;
#105905=ADVANCED_FACE ( 'NONE', ( #56778 ), #47638, .T. ) ;
#105906=CONICAL_SURFACE ( 'NONE', #32776, 0.09999999999999982514, 0.003490658503988666988 ) ;
#105907=EDGE_CURVE ( 'NONE', #14967, #51095, #47000, .T. ) ;
#105908=ORIENTED_EDGE ( 'NONE', *, *, #88728, .T. ) ;
#105909=ADVANCED_FACE ( 'NONE', ( #38483 ), #37822, .T. ) ;
#105910=AXIS2_PLACEMENT_3D ( 'NONE', #78963, #119501, #60613 ) ;
#105911=CIRCLE ( 'NONE', #49404, 0.09999999999999982514 ) ;
#105912=EDGE_CURVE ( 'NONE', #80364, #73565, #67232, .T. ) ;
#105913=EDGE_LOOP ( 'NONE', ( #6343, #100617 ) ) ;
#105914=ORIENTED_EDGE ( 'NONE', *, *, #16617, .F. ) ;
#105915=CARTESIAN_POINT ( 'NONE',  ( -13.74999999999998757, 2.500000000000000000, -2.757883832488651876 ) ) ;
#105916=DIRECTION ( 'NONE',  ( -4.274815082592931898E-19, -0.9999939076577903929, -0.003490651415223739937 ) ) ;
#105917=DIRECTION ( 'NONE',  ( -0.000000000000000000, -1.000000000000000000, -0.000000000000000000 ) ) ;
#105918=FACE_BOUND ( 'NONE', #113428, .T. ) ;
#105919=CARTESIAN_POINT ( 'NONE',  ( 2.899999999999946620, 2.500000000000000000, -0.5928203230275542746 ) ) ;
#105920=DIRECTION ( 'NONE',  ( 0.000000000000000000, 1.000000000000000000, 0.000000000000000000 ) ) ;
#105921=EDGE_CURVE ( 'NONE', #71628, #7939, #78401, .T. ) ;
#105922=CARTESIAN_POINT ( 'NONE',  ( 14.39999999999989555, 2.500000000000000000, -0.3464101615137782364 ) ) ;
#105923=DIRECTION ( 'NONE',  ( 0.000000000000000000, 0.000000000000000000, 1.000000000000000000 ) ) ;
#105925=DIRECTION ( 'NONE',  ( 0.000000000000000000, 0.000000000000000000, 1.000000000000000000 ) ) ;
#105926=DIRECTION ( 'NONE',  ( 0.000000000000000000, 0.000000000000000000, 1.000000000000000000 ) ) ;
#105927=CARTESIAN_POINT ( 'NONE',  ( -1.250000000000001110, 2.500000000000000000, -6.395190528383301931 ) ) ;
#105928=VERTEX_POINT ( 'NONE', #107841 ) ;
#105929=ORIENTED_EDGE ( 'NONE', *, *, #70582, .T. ) ;
#105930=VERTEX_POINT ( 'NONE', #18165 ) ;
#105931=EDGE_LOOP ( 'NONE', ( #82255, #52021, #124619, #127540 ) ) ;
#105932=DIRECTION ( 'NONE',  ( 0.000000000000000000, 0.000000000000000000, 1.000000000000000000 ) ) ;
#105933=EDGE_CURVE ( 'NONE', #38823, #80116, #8343, .T. ) ;
#105934=FACE_BOUND ( 'NONE', #18523, .T. ) ;
#105935=FACE_OUTER_BOUND ( 'NONE', #68887, .T. ) ;
#105936=CIRCLE ( 'NONE', #34858, 0.1000000000000002554 ) ;
#105937=CONICAL_SURFACE ( 'NONE', #55844, 0.1000000000000000472, 0.003490658503988666988 ) ;
#105938=ORIENTED_EDGE ( 'NONE', *, *, #62297, .T. ) ;
#105939=CARTESIAN_POINT ( 'NONE',  ( 11.64999999999990443, 12.50000000000000000, 1.472243186433545459 ) ) ;
#105940=CARTESIAN_POINT ( 'NONE',  ( 0.5999999999999555689, 12.50000000000000000, 4.676537180435972552 ) ) ;
#105941=EDGE_LOOP ( 'NONE', ( #99747, #118476 ) ) ;
#105943=CARTESIAN_POINT ( 'NONE',  ( -10.45000000000000462, 2.500000000000000000, -2.065063509461098068 ) ) ;
#105944=CONICAL_SURFACE ( 'NONE', #66226, 0.09999999999999982514, 0.003490658503988666988 ) ;
#105945=CIRCLE ( 'NONE', #9802, 0.06509327318403745899 ) ;
#105946=EDGE_CURVE ( 'NONE', #73985, #92776, #79591, .T. ) ;
#105947=ORIENTED_EDGE ( 'NONE', *, *, #90454, .T. ) ;
#105948=FACE_OUTER_BOUND ( 'NONE', #36916, .T. ) ;
#105949=CARTESIAN_POINT ( 'NONE',  ( -12.69999999999999396, 2.500000000000000000, -4.083716857408424161 ) ) ;
#105950=CONICAL_SURFACE ( 'NONE', #22347, 0.1000000000000000056, 0.003490658503988666988 ) ;
#105951=AXIS2_PLACEMENT_3D ( 'NONE', #62257, #63538, #12491 ) ;
#105952=AXIS2_PLACEMENT_3D ( 'NONE', #41230, #20278, #40598 ) ;
#105953=EDGE_LOOP ( 'NONE', ( #114917, #13554, #110158, #40690 ) ) ;
#105954=AXIS2_PLACEMENT_3D ( 'NONE', #110916, #111576, #110286 ) ;
#105955=CARTESIAN_POINT ( 'NONE',  ( 8.099999999999921485, 12.50000000000000000, -0.2813168883297409439 ) ) ;
#105956=DIRECTION ( 'NONE',  ( 0.000000000000000000, 1.000000000000000000, 0.000000000000000000 ) ) ;
#105957=ORIENTED_EDGE ( 'NONE', *, *, #98418, .F. ) ;
#105958=DIRECTION ( 'NONE',  ( -0.000000000000000000, 1.000000000000000000, -0.000000000000000000 ) ) ;
#105959=ORIENTED_EDGE ( 'NONE', *, *, #4892, .T. ) ;
#105960=ORIENTED_EDGE ( 'NONE', *, *, #35577, .F. ) ;
#105961=EDGE_CURVE ( 'NONE', #92955, #46558, #42027, .T. ) ;
#105962=PLANE ( 'NONE',  #43133 ) ;
#105963=ORIENTED_EDGE ( 'NONE', *, *, #46467, .T. ) ;
#105964=CARTESIAN_POINT ( 'NONE',  ( 5.199999999999935341, 12.50000000000000000, -0.3464101615137783474 ) ) ;
#105965=CARTESIAN_POINT ( 'NONE',  ( -0.4500000000000402012, 2.500000000000000000, 2.065063509461097624 ) ) ;
#105966=VERTEX_POINT ( 'NONE', #22056 ) ;
#105967=DIRECTION ( 'NONE',  ( -0.000000000000000000, 1.000000000000000000, -0.000000000000000000 ) ) ;
#105968=CARTESIAN_POINT ( 'NONE',  ( 8.949999999999915801, 12.50000000000000000, -1.753560074763288679 ) ) ;
#105969=FACE_OUTER_BOUND ( 'NONE', #79272, .T. ) ;
#105970=CARTESIAN_POINT ( 'NONE',  ( 6.049999999999934097, 2.500000000000000000, -6.148780366869526226 ) ) ;
#105971=DIRECTION ( 'NONE',  ( 0.000000000000000000, 0.000000000000000000, -1.000000000000000000 ) ) ;
#105972=CONICAL_SURFACE ( 'NONE', #24410, 0.09999999999999982514, 0.003490658503988666988 ) ;
#105973=CARTESIAN_POINT ( 'NONE',  ( 17.41716098457701634, 1.872967139268043146, -4.643356076170611857 ) ) ;
#105975=VECTOR ( 'NONE', #21782, 1000.000000000000000 ) ;
#105976=EDGE_LOOP ( 'NONE', ( #78076, #123138 ) ) ;
#105977=VERTEX_POINT ( 'NONE', #112357 ) ;
#105978=CARTESIAN_POINT ( 'NONE',  ( -2.300000000000033573, 2.500000000000000000, -4.083716857408426826 ) ) ;
#105979=AXIS2_PLACEMENT_3D ( 'NONE', #45393, #46673, #55212 ) ;
#105980=DIRECTION ( 'NONE',  ( 0.000000000000000000, 0.000000000000000000, 1.000000000000000000 ) ) ;
#105981=CARTESIAN_POINT ( 'NONE',  ( 0.8499999999999557909, 12.50000000000000000, -6.560283801567339701 ) ) ;
#105982=EDGE_LOOP ( 'NONE', ( #11557, #67078 ) ) ;
#105984=ORIENTED_EDGE ( 'NONE', *, *, #109057, .F. ) ;
#105985=FACE_OUTER_BOUND ( 'NONE', #116694, .T. ) ;
#105986=AXIS2_PLACEMENT_3D ( 'NONE', #105787, #27870, #126720 ) ;
#105987=CONICAL_SURFACE ( 'NONE', #30702, 0.09999999999999982514, 0.003490658503988666988 ) ;
#105988=DIRECTION ( 'NONE',  ( 0.000000000000000000, 0.000000000000000000, -1.000000000000000000 ) ) ;
#105989=DIRECTION ( 'NONE',  ( 0.000000000000000000, 0.000000000000000000, -1.000000000000000000 ) ) ;
#105990=CONICAL_SURFACE ( 'NONE', #114297, 0.1000000000000000056, 0.003490658503988666988 ) ;
#105991=EDGE_CURVE ( 'NONE', #18296, #118526, #52477, .T. ) ;
#105993=CARTESIAN_POINT ( 'NONE',  ( 4.399999999999937295, 2.500000000000000000, 3.983716857408420964 ) ) ;
#105994=CARTESIAN_POINT ( 'NONE',  ( 6.049999999999930544, 12.50000000000000000, 2.511473670974873507 ) ) ;
#105995=CARTESIAN_POINT ( 'NONE',  ( -13.29999999999999005, 2.500000000000000000, 1.843143693225357538E-15 ) ) ;
#105996=DIRECTION ( 'NONE',  ( 0.000000000000000000, 1.000000000000000000, 0.000000000000000000 ) ) ;
#105997=CARTESIAN_POINT ( 'NONE',  ( -3.150000000000033218, 2.500000000000000000, -6.841600689897078702 ) ) ;
#105999=FACE_OUTER_BOUND ( 'NONE', #102674, .T. ) ;
#106000=CIRCLE ( 'NONE', #91327, 0.06509327318403745899 ) ;
#106001=ORIENTED_EDGE ( 'NONE', *, *, #67390, .F. ) ;
#106002=VECTOR ( 'NONE', #62541, 1000.000000000000000 ) ;
#106003=CIRCLE ( 'NONE', #122728, 0.1000000000000002554 ) ;
#106004=DIRECTION ( 'NONE',  ( 0.000000000000000000, 0.000000000000000000, 1.000000000000000000 ) ) ;
#106006=VERTEX_POINT ( 'NONE', #50227 ) ;
#106007=EDGE_CURVE ( 'NONE', #17553, #119696, #87971, .T. ) ;
#106008=ORIENTED_EDGE ( 'NONE', *, *, #116165, .F. ) ;
#106009=EDGE_CURVE ( 'NONE', #37406, #11230, #1739, .T. ) ;
#106010=DIRECTION ( 'NONE',  ( 0.000000000000000000, 1.000000000000000000, 0.000000000000000000 ) ) ;
#106011=LINE ( 'NONE', #76549, #69810 ) ;
#106012=EDGE_CURVE ( 'NONE', #26373, #100348, #56583, .T. ) ;
#106013=DIRECTION ( 'NONE',  ( 0.000000000000000000, 0.000000000000000000, -1.000000000000000000 ) ) ;
#106014=CARTESIAN_POINT ( 'NONE',  ( 1.899999999999951283, 2.500000000000000000, 0.3464101615137736845 ) ) ;
#106015=CARTESIAN_POINT ( 'NONE',  ( -2.700000000000029932, 12.50000000000000000, -4.676537180435977881 ) ) ;
#106016=DIRECTION ( 'NONE',  ( -0.000000000000000000, 1.000000000000000000, -0.000000000000000000 ) ) ;
#106017=CARTESIAN_POINT ( 'NONE',  ( 5.849999999999933920, 12.50000000000000000, -2.922977105672691422 ) ) ;
#106018=ORIENTED_EDGE ( 'NONE', *, *, #81654, .T. ) ;
#106019=CARTESIAN_POINT ( 'NONE',  ( -6.250000000000017764, 2.500000000000000000, 2.857883832488649301 ) ) ;
#106020=ADVANCED_FACE ( 'NONE', ( #33164 ), #102526, .T. ) ;
#106021=CARTESIAN_POINT ( 'NONE',  ( -12.94999999999999218, 2.500000000000000000, -2.265063509461099578 ) ) ;
#106022=EDGE_CURVE ( 'NONE', #4486, #11304, #58757, .T. ) ;
#106023=ORIENTED_EDGE ( 'NONE', *, *, #44728, .F. ) ;
#106024=EDGE_CURVE ( 'NONE', #34064, #35601, #125634, .T. ) ;
#106025=ORIENTED_EDGE ( 'NONE', *, *, #3334, .T. ) ;
#106027=EDGE_LOOP ( 'NONE', ( #16824, #88620 ) ) ;
#106028=DIRECTION ( 'NONE',  ( 0.000000000000000000, -0.9999939076577903929, 0.003490651415223739937 ) ) ;
#106029=DIRECTION ( 'NONE',  ( 0.000000000000000000, 0.000000000000000000, -1.000000000000000000 ) ) ;
#106030=CONICAL_SURFACE ( 'NONE', #103882, 0.09999999999999999167, 0.003490658503988666988 ) ;
#106031=CARTESIAN_POINT ( 'NONE',  ( -12.04999999999999538, 12.50000000000000000, 6.430097255199259010 ) ) ;
#106032=AXIS2_PLACEMENT_3D ( 'NONE', #29738, #90582, #17975 ) ;
#106033=DIRECTION ( 'NONE',  ( 0.000000000000000000, 0.000000000000000000, 1.000000000000000000 ) ) ;
#106034=DIRECTION ( 'NONE',  ( 0.000000000000000000, -0.000000000000000000, 1.000000000000000000 ) ) ;
#106035=ORIENTED_EDGE ( 'NONE', *, *, #98475, .T. ) ;
#106036=DIRECTION ( 'NONE',  ( -4.274815082592931898E-19, -0.9999939076577903929, -0.003490651415223739937 ) ) ;
#106037=CIRCLE ( 'NONE', #89312, 0.06509327318403745899 ) ;
#106038=DIRECTION ( 'NONE',  ( 0.000000000000000000, 0.000000000000000000, 1.000000000000000000 ) ) ;
#106039=ORIENTED_EDGE ( 'NONE', *, *, #53365, .F. ) ;
#106040=CONICAL_SURFACE ( 'NONE', #74746, 0.09999999999999982514, 0.003490658503988666988 ) ;
#106041=ORIENTED_EDGE ( 'NONE', *, *, #30964, .T. ) ;
#106042=VERTEX_POINT ( 'NONE', #111709 ) ;
#106043=CARTESIAN_POINT ( 'NONE',  ( -6.250000000000019540, 2.500000000000000000, -7.088010851410853519 ) ) ;
#106044=CIRCLE ( 'NONE', #87162, 0.1000000000000002554 ) ;
#106045=DIRECTION ( 'NONE',  ( 0.000000000000000000, 0.000000000000000000, -1.000000000000000000 ) ) ;
#106046=CARTESIAN_POINT ( 'NONE',  ( -9.350000000000006750, 12.50000000000000000, 1.818653347947321475 ) ) ;
#106047=VECTOR ( 'NONE', #70211, 1000.000000000000000 ) ;
#106048=ORIENTED_EDGE ( 'NONE', *, *, #20340, .T. ) ;
#106049=FACE_OUTER_BOUND ( 'NONE', #69577, .T. ) ;
#106050=DIRECTION ( 'NONE',  ( 0.000000000000000000, 0.000000000000000000, 1.000000000000000000 ) ) ;
#106051=CARTESIAN_POINT ( 'NONE',  ( -12.49999999999999289, 2.500000000000000000, 3.637306695894644726 ) ) ;
#106052=DIRECTION ( 'NONE',  ( 0.000000000000000000, 1.000000000000000000, 0.000000000000000000 ) ) ;
#106053=ADVANCED_FACE ( 'NONE', ( #1102 ), #41697, .T. ) ;
#106054=FACE_OUTER_BOUND ( 'NONE', #55393, .T. ) ;
#106055=ADVANCED_FACE ( 'NONE', ( #3053 ), #31564, .T. ) ;
#106056=VERTEX_POINT ( 'NONE', #80326 ) ;
#106057=AXIS2_PLACEMENT_3D ( 'NONE', #104966, #36265, #75515 ) ;
#106058=CARTESIAN_POINT ( 'NONE',  ( -7.050000000000013145, 12.50000000000000000, 2.230156782645134950 ) ) ;
#106059=EDGE_CURVE ( 'NONE', #16889, #127557, #30591, .T. ) ;
#106060=ORIENTED_EDGE ( 'NONE', *, *, #19780, .T. ) ;
#106061=VERTEX_POINT ( 'NONE', #81597 ) ;
#106062=EDGE_LOOP ( 'NONE', ( #31727, #95114, #113145, #67005 ) ) ;
#106063=DIRECTION ( 'NONE',  ( -4.274815082592931898E-19, -0.9999939076577903929, -0.003490651415223739937 ) ) ;
#106064=FACE_BOUND ( 'NONE', #73209, .T. ) ;
#106065=AXIS2_PLACEMENT_3D ( 'NONE', #41117, #100641, #120937 ) ;
#106066=CARTESIAN_POINT ( 'NONE',  ( -8.550000000000011369, 2.500000000000000000, 1.718653347947321386 ) ) ;
#106067=CARTESIAN_POINT ( 'NONE',  ( -4.150000000000025224, 2.500000000000000000, 5.802370205355744659 ) ) ;
#106068=AXIS2_PLACEMENT_3D ( 'NONE', #120457, #42564, #1957 ) ;
#106069=ADVANCED_FACE ( 'NONE', ( #20750 ), #123489, .T. ) ;
#106070=CARTESIAN_POINT ( 'NONE',  ( 3.149999999999946176, 12.50000000000000000, -2.446380397790840266 ) ) ;
#106071=CIRCLE ( 'NONE', #53847, 0.09999999999999982514 ) ;
#106072=ORIENTED_EDGE ( 'NONE', *, *, #109584, .T. ) ;
#106074=DIRECTION ( 'NONE',  ( 0.000000000000000000, 0.000000000000000000, 1.000000000000000000 ) ) ;
#106075=CONICAL_SURFACE ( 'NONE', #93471, 0.1000000000000000056, 0.003490658503988666988 ) ;
#106076=DIRECTION ( 'NONE',  ( 0.000000000000000000, 0.000000000000000000, -1.000000000000000000 ) ) ;
#106078=CARTESIAN_POINT ( 'NONE',  ( -1.450000000000036371, 2.500000000000000000, 2.511473670974873507 ) ) ;
#106079=EDGE_LOOP ( 'NONE', ( #48000, #37388 ) ) ;
#106080=DIRECTION ( 'NONE',  ( 0.000000000000000000, 0.000000000000000000, 1.000000000000000000 ) ) ;
#106081=AXIS2_PLACEMENT_3D ( 'NONE', #35987, #15680, #115831 ) ;
#106082=CIRCLE ( 'NONE', #127022, 0.06509327318403745899 ) ;
#106083=FACE_OUTER_BOUND ( 'NONE', #50392, .T. ) ;
#106084=ORIENTED_EDGE ( 'NONE', *, *, #103781, .T. ) ;
#106085=CARTESIAN_POINT ( 'NONE',  ( 5.599999999999931255, 2.500000000000000000, 4.776537180435972196 ) ) ;
#106086=AXIS2_PLACEMENT_3D ( 'NONE', #9059, #77165, #20176 ) ;
#106087=FACE_BOUND ( 'NONE', #9533, .T. ) ;
#106089=AXIS2_PLACEMENT_3D ( 'NONE', #124018, #14047, #37591 ) ;
#106090=AXIS2_PLACEMENT_3D ( 'NONE', #92771, #103874, #62668 ) ;
#106091=VERTEX_POINT ( 'NONE', #90772 ) ;
#106093=FACE_OUTER_BOUND ( 'NONE', #103894, .T. ) ;
#106094=ORIENTED_EDGE ( 'NONE', *, *, #88398, .T. ) ;
#106095=ORIENTED_EDGE ( 'NONE', *, *, #1557, .T. ) ;
#106097=ORIENTED_EDGE ( 'NONE', *, *, #27200, .F. ) ;
#106099=CARTESIAN_POINT ( 'NONE',  ( -4.350000000000023626, 2.500000000000000000, 6.841600689897072485 ) ) ;
#106100=EDGE_CURVE ( 'NONE', #9122, #105841, #46137, .T. ) ;
#106101=DIRECTION ( 'NONE',  ( 0.000000000000000000, 0.000000000000000000, 1.000000000000000000 ) ) ;
#106102=CARTESIAN_POINT ( 'NONE',  ( -8.550000000000011369, 2.500000000000000000, 1.818653347947321475 ) ) ;
#106103=DIRECTION ( 'NONE',  ( 0.000000000000000000, 0.000000000000000000, 1.000000000000000000 ) ) ;
#106104=AXIS2_PLACEMENT_3D ( 'NONE', #36857, #67573, #117972 ) ;
#106105=EDGE_LOOP ( 'NONE', ( #110760, #24206, #116992, #31936 ) ) ;
#106106=DIRECTION ( 'NONE',  ( 0.000000000000000000, 1.000000000000000000, 0.000000000000000000 ) ) ;
#106107=CARTESIAN_POINT ( 'NONE',  ( 9.999999999999912959, 2.500000000000000000, 3.737306695894644371 ) ) ;
#106108=DIRECTION ( 'NONE',  ( 0.000000000000000000, -0.9999939076577903929, 0.003490651415223739937 ) ) ;
#106109=ADVANCED_FACE ( 'NONE', ( #71131 ), #111036, .T. ) ;
#106111=VERTEX_POINT ( 'NONE', #3683 ) ;
#106112=EDGE_LOOP ( 'NONE', ( #75996, #78022 ) ) ;
#106113=FACE_BOUND ( 'NONE', #49192, .T. ) ;
#106114=ORIENTED_EDGE ( 'NONE', *, *, #110114, .F. ) ;
#106115=EDGE_CURVE ( 'NONE', #95740, #38693, #119286, .T. ) ;
#106116=DIRECTION ( 'NONE',  ( 0.000000000000000000, 1.000000000000000000, 0.000000000000000000 ) ) ;
#106117=DIRECTION ( 'NONE',  ( 0.000000000000000000, 0.000000000000000000, -1.000000000000000000 ) ) ;
#106118=EDGE_LOOP ( 'NONE', ( #112724, #67981, #16323, #69576 ) ) ;
#106119=PLANE ( 'NONE',  #78600 ) ;
#106120=CARTESIAN_POINT ( 'NONE',  ( 7.949999999999922018, 12.50000000000000000, 6.430097255199259010 ) ) ;
#106121=FACE_OUTER_BOUND ( 'NONE', #34846, .T. ) ;
#106122=CIRCLE ( 'NONE', #24554, 0.06509327318403745899 ) ;
#106123=CARTESIAN_POINT ( 'NONE',  ( 9.199999999999915801, 12.50000000000000000, -4.265033745738164406 ) ) ;
#106124=ORIENTED_EDGE ( 'NONE', *, *, #38690, .F. ) ;
#106125=FACE_OUTER_BOUND ( 'NONE', #120374, .T. ) ;
#106126=LINE ( 'NONE', #56372, #60647 ) ;
#106127=EDGE_CURVE ( 'NONE', #29957, #22780, #102559, .T. ) ;
#106129=DIRECTION ( 'NONE',  ( 0.000000000000000000, 1.000000000000000000, 0.000000000000000000 ) ) ;
#106130=CARTESIAN_POINT ( 'NONE',  ( -9.400000000000007461, 12.50000000000000000, 3.983716857408420076 ) ) ;
#106131=VERTEX_POINT ( 'NONE', #55995 ) ;
#106132=AXIS2_PLACEMENT_3D ( 'NONE', #111443, #41453, #120635 ) ;
#106133=AXIS2_PLACEMENT_3D ( 'NONE', #79821, #47793, #128951 ) ;
#106134=ORIENTED_EDGE ( 'NONE', *, *, #1288, .F. ) ;
#106136=VERTEX_POINT ( 'NONE', #65157 ) ;
#106137=CARTESIAN_POINT ( 'NONE',  ( 6.849999999999930367, 12.50000000000000000, -6.148780366869526226 ) ) ;
#106138=ORIENTED_EDGE ( 'NONE', *, *, #125767, .T. ) ;
#106139=ORIENTED_EDGE ( 'NONE', *, *, #112731, .F. ) ;
#106141=CARTESIAN_POINT ( 'NONE',  ( -8.350000000000013856, 2.500000000000000000, 2.165063509461097713 ) ) ;
#106142=VECTOR ( 'NONE', #118496, 1000.000000000000000 ) ;
#106143=CARTESIAN_POINT ( 'NONE',  ( 13.74999999999989342, 2.500000000000000000, -1.372243186433550033 ) ) ;
#106144=DIRECTION ( 'NONE',  ( 0.000000000000000000, 0.000000000000000000, -1.000000000000000000 ) ) ;
#106145=ADVANCED_FACE ( 'NONE', ( #53446 ), #54525, .T. ) ;
#106146=FACE_OUTER_BOUND ( 'NONE', #60231, .T. ) ;
#106147=LINE ( 'NONE', #85846, #8276 ) ;
#106148=DIRECTION ( 'NONE',  ( 0.000000000000000000, 0.000000000000000000, 1.000000000000000000 ) ) ;
#106149=AXIS2_PLACEMENT_3D ( 'NONE', #116792, #18604, #58548 ) ;
#106151=CARTESIAN_POINT ( 'NONE',  ( -13.09999999999999076, 12.50000000000000000, 3.983716857408420964 ) ) ;
#106152=ORIENTED_EDGE ( 'NONE', *, *, #95508, .T. ) ;
#106153=EDGE_CURVE ( 'NONE', #90081, #80887, #105088, .T. ) ;
#106154=AXIS2_PLACEMENT_3D ( 'NONE', #75797, #66624, #7049 ) ;
#106155=ORIENTED_EDGE ( 'NONE', *, *, #1546, .F. ) ;
#106156=EDGE_LOOP ( 'NONE', ( #19743, #59685, #104220, #14319 ) ) ;
#106157=ORIENTED_EDGE ( 'NONE', *, *, #8467, .F. ) ;
#106158=AXIS2_PLACEMENT_3D ( 'NONE', #111607, #122082, #72346 ) ;
#106159=CARTESIAN_POINT ( 'NONE',  ( 2.099999999999949463, 2.500000000000000000, -3.537306695894649966 ) ) ;
#106160=EDGE_CURVE ( 'NONE', #48527, #12263, #113029, .T. ) ;
#106161=ORIENTED_EDGE ( 'NONE', *, *, #68193, .F. ) ;
#106162=ADVANCED_FACE ( 'NONE', ( #55368 ), #67041, .T. ) ;
#106163=VERTEX_POINT ( 'NONE', #103826 ) ;
#106164=EDGE_CURVE ( 'NONE', #93502, #50283, #114276, .T. ) ;
#106165=AXIS2_PLACEMENT_3D ( 'NONE', #67003, #57859, #58514 ) ;
#106166=ADVANCED_FACE ( 'NONE', ( #95292 ), #35726, .T. ) ;
#106168=CARTESIAN_POINT ( 'NONE',  ( -2.900000000000029221, 12.50000000000000000, -4.957854068765716882 ) ) ;
#106169=DIRECTION ( 'NONE',  ( 0.000000000000000000, 0.000000000000000000, 1.000000000000000000 ) ) ;
#106170=VECTOR ( 'NONE', #74824, 1000.000000000000000 ) ;
#106171=DIRECTION ( 'NONE',  ( 0.000000000000000000, 1.000000000000000000, 0.000000000000000000 ) ) ;
#106172=CARTESIAN_POINT ( 'NONE',  ( 6.849999999999930367, 2.500000000000000000, -6.841600689897078702 ) ) ;
#106173=EDGE_CURVE ( 'NONE', #115875, #60164, #117208, .T. ) ;
#106174=CARTESIAN_POINT ( 'NONE',  ( 8.299999999999922551, 2.500000000000000000, 4.330127018922196314 ) ) ;
#106175=EDGE_LOOP ( 'NONE', ( #76232, #67683 ) ) ;
#106176=EDGE_CURVE ( 'NONE', #127833, #82531, #85463, .T. ) ;
#106177=VECTOR ( 'NONE', #129172, 1000.000000000000000 ) ;
#106178=CARTESIAN_POINT ( 'NONE',  ( -2.900000000000029221, 2.500000000000000000, 0.09999999999999772959 ) ) ;
#106179=ADVANCED_FACE ( 'NONE', ( #83546 ), #121434, .T. ) ;
#106180=EDGE_LOOP ( 'NONE', ( #86490, #127339, #41464, #41741 ) ) ;
#106181=AXIS2_PLACEMENT_3D ( 'NONE', #117619, #75784, #128123 ) ;
#106182=DIRECTION ( 'NONE',  ( -4.274815082592931898E-19, -0.9999939076577903929, -0.003490651415223739937 ) ) ;
#106183=EDGE_CURVE ( 'NONE', #16039, #84307, #94251, .T. ) ;
#106184=ORIENTED_EDGE ( 'NONE', *, *, #23535, .T. ) ;
#106185=DIRECTION ( 'NONE',  ( 0.000000000000000000, 0.000000000000000000, 1.000000000000000000 ) ) ;
#106186=ORIENTED_EDGE ( 'NONE', *, *, #3868, .F. ) ;
#106187=AXIS2_PLACEMENT_3D ( 'NONE', #78960, #119500, #96624 ) ;
#106188=ORIENTED_EDGE ( 'NONE', *, *, #62246, .F. ) ;
#106189=EDGE_CURVE ( 'NONE', #104360, #52455, #247, .T. ) ;
#106190=CARTESIAN_POINT ( 'NONE',  ( -9.350000000000006750, 12.50000000000000000, 2.511473670974873507 ) ) ;
#106191=FACE_OUTER_BOUND ( 'NONE', #35300, .T. ) ;
#106192=AXIS2_PLACEMENT_3D ( 'NONE', #102935, #112129, #51289 ) ;
#106193=CARTESIAN_POINT ( 'NONE',  ( -4.150000000000024336, 2.500000000000000000, -2.857883832488653741 ) ) ;
#106195=DIRECTION ( 'NONE',  ( 0.000000000000000000, 1.000000000000000000, 0.000000000000000000 ) ) ;
#106196=ORIENTED_EDGE ( 'NONE', *, *, #113835, .T. ) ;
#106197=DIRECTION ( 'NONE',  ( 0.000000000000000000, 0.000000000000000000, -1.000000000000000000 ) ) ;
#106198=CARTESIAN_POINT ( 'NONE',  ( 8.749999999999920064, 12.50000000000000000, -2.792790559304616504 ) ) ;
#106199=DIRECTION ( 'NONE',  ( -0.000000000000000000, -1.000000000000000000, -0.000000000000000000 ) ) ;
#106200=CARTESIAN_POINT ( 'NONE',  ( 12.49999999999990230, 12.50000000000000000, -0.6928203230275541413 ) ) ;
#106201=DIRECTION ( 'NONE',  ( -0.000000000000000000, -1.000000000000000000, -0.000000000000000000 ) ) ;
#106202=EDGE_LOOP ( 'NONE', ( #55297, #26255 ) ) ;
#106203=ORIENTED_EDGE ( 'NONE', *, *, #15112, .F. ) ;
#106204=LINE ( 'NONE', #26361, #113292 ) ;
#106205=ORIENTED_EDGE ( 'NONE', *, *, #89942, .T. ) ;
#106206=DIRECTION ( 'NONE',  ( 0.000000000000000000, 1.000000000000000000, 0.000000000000000000 ) ) ;
#106207=DIRECTION ( 'NONE',  ( 0.000000000000000000, 1.000000000000000000, 0.000000000000000000 ) ) ;
#106208=AXIS2_PLACEMENT_3D ( 'NONE', #10488, #20327, #119810 ) ;
#106209=CIRCLE ( 'NONE', #49790, 0.09999999999999982514 ) ;
#106210=ORIENTED_EDGE ( 'NONE', *, *, #44438, .F. ) ;
#106212=LINE ( 'NONE', #97672, #91232 ) ;
#106213=CARTESIAN_POINT ( 'NONE',  ( -10.65000000000000213, 2.500000000000000000, 1.818653347947321475 ) ) ;
#106214=CARTESIAN_POINT ( 'NONE',  ( 2.499999999999947153, 2.500000000000000000, 3.537306695894645081 ) ) ;
#106215=ORIENTED_EDGE ( 'NONE', *, *, #62137, .T. ) ;
#106216=CONICAL_SURFACE ( 'NONE', #108266, 0.1000000000000002554, 0.003490658503988666988 ) ;
#106217=EDGE_CURVE ( 'NONE', #109827, #127552, #112995, .T. ) ;
#106218=CIRCLE ( 'NONE', #74822, 0.1000000000000002554 ) ;
#106219=DIRECTION ( 'NONE',  ( -0.000000000000000000, 1.000000000000000000, -0.000000000000000000 ) ) ;
#106220=CARTESIAN_POINT ( 'NONE',  ( 7.099999999999928590, 12.50000000000000000, 4.395220292106234439 ) ) ;
#106221=ADVANCED_FACE ( 'NONE', ( #73699 ), #4296, .T. ) ;
#106222=ORIENTED_EDGE ( 'NONE', *, *, #116970, .F. ) ;
#106223=DIRECTION ( 'NONE',  ( 0.000000000000000000, 0.000000000000000000, 1.000000000000000000 ) ) ;
#106224=DIRECTION ( 'NONE',  ( -0.000000000000000000, -1.000000000000000000, -0.000000000000000000 ) ) ;
#106225=CIRCLE ( 'NONE', #97895, 0.09999999999999982514 ) ;
#106226=CARTESIAN_POINT ( 'NONE',  ( -8.550000000000007816, 2.500000000000000000, 6.248780366869520542 ) ) ;
#106227=VECTOR ( 'NONE', #608, 1000.000000000000000 ) ;
#106228=ORIENTED_EDGE ( 'NONE', *, *, #42323, .F. ) ;
#106229=DIRECTION ( 'NONE',  ( 0.000000000000000000, 1.000000000000000000, 0.000000000000000000 ) ) ;
#106230=EDGE_LOOP ( 'NONE', ( #37639, #107185, #107426, #58834 ) ) ;
#106231=DIRECTION ( 'NONE',  ( 0.000000000000000000, 1.000000000000000000, 0.000000000000000000 ) ) ;
#106232=CARTESIAN_POINT ( 'NONE',  ( -8.550000000000013145, 2.500000000000000000, -6.841600689897073373 ) ) ;
#106233=CARTESIAN_POINT ( 'NONE',  ( -8.950000000000006395, 2.500000000000000000, 6.841600689897072485 ) ) ;
#106234=ORIENTED_EDGE ( 'NONE', *, *, #72212, .T. ) ;
#106235=AXIS2_PLACEMENT_3D ( 'NONE', #84381, #43192, #33371 ) ;
#106236=CARTESIAN_POINT ( 'NONE',  ( 3.349999999999941025, 2.500000000000000000, 7.188010851410848723 ) ) ;
#106237=FACE_OUTER_BOUND ( 'NONE', #95258, .T. ) ;
#106238=CIRCLE ( 'NONE', #49826, 0.09999999999999999167 ) ;
#106239=VERTEX_POINT ( 'NONE', #74360 ) ;
#106241=DIRECTION ( 'NONE',  ( -0.000000000000000000, -1.000000000000000000, -0.000000000000000000 ) ) ;
#106242=ORIENTED_EDGE ( 'NONE', *, *, #112253, .T. ) ;
#106244=CARTESIAN_POINT ( 'NONE',  ( 3.749999999999944045, 2.500000000000000000, -2.757883832488654097 ) ) ;
#106245=FACE_OUTER_BOUND ( 'NONE', #77979, .T. ) ;
#106246=ORIENTED_EDGE ( 'NONE', *, *, #30277, .T. ) ;
#106247=DIRECTION ( 'NONE',  ( -4.274815082592931898E-19, -0.9999939076577903929, -0.003490651415223739937 ) ) ;
#106248=CARTESIAN_POINT ( 'NONE',  ( 10.44999999999991047, 12.50000000000000000, 2.165063509461097713 ) ) ;
#106249=AXIS2_PLACEMENT_3D ( 'NONE', #16295, #5833, #24852 ) ;
#106250=ORIENTED_EDGE ( 'NONE', *, *, #61977, .T. ) ;
#106251=DIRECTION ( 'NONE',  ( -0.000000000000000000, -1.000000000000000000, -0.000000000000000000 ) ) ;
#106252=ADVANCED_FACE ( 'NONE', ( #104458 ), #127792, .T. ) ;
#106253=DIRECTION ( 'NONE',  ( 0.000000000000000000, 0.000000000000000000, -1.000000000000000000 ) ) ;
#106254=CONICAL_SURFACE ( 'NONE', #62357, 0.1000000000000000472, 0.003490658503988666988 ) ;
#106255=FACE_OUTER_BOUND ( 'NONE', #87637, .T. ) ;
#106256=CARTESIAN_POINT ( 'NONE',  ( 12.89999999999990266, 12.50000000000000000, 5.022947341949748790 ) ) ;
#106257=CARTESIAN_POINT ( 'NONE',  ( 10.64999999999990976, 2.500000000000000000, -6.048780366869526581 ) ) ;
#106259=VERTEX_POINT ( 'NONE', #114912 ) ;
#106260=EDGE_LOOP ( 'NONE', ( #49873, #22505, #80094, #60680 ) ) ;
#106261=ORIENTED_EDGE ( 'NONE', *, *, #26232, .T. ) ;
#106262=VERTEX_POINT ( 'NONE', #84815 ) ;
#106263=DIRECTION ( 'NONE',  ( -0.000000000000000000, 1.000000000000000000, -0.000000000000000000 ) ) ;
#106264=DIRECTION ( 'NONE',  ( 0.000000000000000000, 1.000000000000000000, 0.000000000000000000 ) ) ;
#106265=ADVANCED_FACE ( 'NONE', ( #88691 ), #90122, .T. ) ;
#106266=CARTESIAN_POINT ( 'NONE',  ( -8.749999999999975131, 12.50000000000000000, -2.165063509461101710 ) ) ;
#106267=AXIS2_PLACEMENT_3D ( 'NONE', #121221, #123780, #42692 ) ;
#106268=EDGE_LOOP ( 'NONE', ( #108582, #97315, #90284, #84588 ) ) ;
#106269=FACE_BOUND ( 'NONE', #93996, .T. ) ;
#106270=EDGE_CURVE ( 'NONE', #107875, #63897, #6477, .T. ) ;
#106271=DIRECTION ( 'NONE',  ( 0.000000000000000000, -0.000000000000000000, 1.000000000000000000 ) ) ;
#106272=DIRECTION ( 'NONE',  ( 0.000000000000000000, 1.000000000000000000, 0.000000000000000000 ) ) ;
#106273=CARTESIAN_POINT ( 'NONE',  ( 9.149999999999920419, 12.50000000000000000, 2.857883832488649301 ) ) ;
#106274=CONICAL_SURFACE ( 'NONE', #35190, 0.1000000000000000472, 0.003490658503988666988 ) ;
#106275=CIRCLE ( 'NONE', #41460, 0.09999999999999982514 ) ;
#106276=FACE_OUTER_BOUND ( 'NONE', #12335, .T. ) ;
#106277=FACE_OUTER_BOUND ( 'NONE', #118776, .T. ) ;
#106278=DIRECTION ( 'NONE',  ( -0.000000000000000000, 1.000000000000000000, -0.000000000000000000 ) ) ;
#106279=CARTESIAN_POINT ( 'NONE',  ( -14.79999999999998295, 2.500000000000000000, -0.3464101615137760715 ) ) ;
#106280=DIRECTION ( 'NONE',  ( 0.000000000000000000, 0.000000000000000000, 1.000000000000000000 ) ) ;
#106281=EDGE_CURVE ( 'NONE', #23602, #64836, #68396, .T. ) ;
#106282=LINE ( 'NONE', #6132, #99629 ) ;
#106283=DIRECTION ( 'NONE',  ( -0.000000000000000000, 1.000000000000000000, -0.000000000000000000 ) ) ;
#106284=ORIENTED_EDGE ( 'NONE', *, *, #85798, .F. ) ;
#106285=EDGE_LOOP ( 'NONE', ( #48933, #115433 ) ) ;
#106286=ORIENTED_EDGE ( 'NONE', *, *, #58873, .F. ) ;
#106287=VERTEX_POINT ( 'NONE', #88015 ) ;
#106288=DIRECTION ( 'NONE',  ( 0.000000000000000000, 1.000000000000000000, 0.000000000000000000 ) ) ;
#106289=AXIS2_PLACEMENT_3D ( 'NONE', #32716, #3869, #74546 ) ;
#106290=DIRECTION ( 'NONE',  ( 0.000000000000000000, 0.000000000000000000, -1.000000000000000000 ) ) ;
#106291=EDGE_LOOP ( 'NONE', ( #47895, #17102 ) ) ;
#106292=ORIENTED_EDGE ( 'NONE', *, *, #105381, .F. ) ;
#106294=CIRCLE ( 'NONE', #66571, 0.06509327318403745899 ) ;
#106295=AXIS2_PLACEMENT_3D ( 'NONE', #120817, #20052, #31169 ) ;
#106296=DIRECTION ( 'NONE',  ( 0.000000000000000000, 1.000000000000000000, 0.000000000000000000 ) ) ;
#106297=VECTOR ( 'NONE', #25319, 1000.000000000000000 ) ;
#106298=DIRECTION ( 'NONE',  ( -0.000000000000000000, -1.000000000000000000, -0.000000000000000000 ) ) ;
#106299=CARTESIAN_POINT ( 'NONE',  ( -11.69999999999999929, 2.500000000000000000, -4.230127018922199333 ) ) ;
#106300=DIRECTION ( 'NONE',  ( -0.000000000000000000, -1.000000000000000000, -0.000000000000000000 ) ) ;
#106301=EDGE_LOOP ( 'NONE', ( #88689, #97680, #110411, #77170 ) ) ;
#106302=CIRCLE ( 'NONE', #70794, 0.1000000000000002554 ) ;
#106303=AXIS2_PLACEMENT_3D ( 'NONE', #20353, #22305, #61580 ) ;
#106304=ORIENTED_EDGE ( 'NONE', *, *, #104282, .T. ) ;
#106305=EDGE_CURVE ( 'NONE', #20680, #55512, #71343, .T. ) ;
#106306=AXIS2_PLACEMENT_3D ( 'NONE', #52873, #2457, #71215 ) ;
#106307=ORIENTED_EDGE ( 'NONE', *, *, #38958, .F. ) ;
#106308=ORIENTED_EDGE ( 'NONE', *, *, #129402, .F. ) ;
#106309=EDGE_LOOP ( 'NONE', ( #46975, #79366 ) ) ;
#106310=EDGE_CURVE ( 'NONE', #25449, #20272, #38984, .T. ) ;
#106311=VERTEX_POINT ( 'NONE', #48776 ) ;
#106312=CONICAL_SURFACE ( 'NONE', #45779, 0.1000000000000000472, 0.003490658503988666988 ) ;
#106313=EDGE_CURVE ( 'NONE', #45263, #6533, #113120, .T. ) ;
#106314=DIRECTION ( 'NONE',  ( -0.000000000000000000, 1.000000000000000000, -0.000000000000000000 ) ) ;
#106316=PLANE ( 'NONE',  #70833 ) ;
#106317=CARTESIAN_POINT ( 'NONE',  ( -6.071532165918824830E-15, 2.500000000000000000, -4.330127018922201643 ) ) ;
#106318=ADVANCED_FACE ( 'NONE', ( #49427 ), #28489, .T. ) ;
#106319=EDGE_CURVE ( 'NONE', #86214, #125645, #29590, .T. ) ;
#106320=CARTESIAN_POINT ( 'NONE',  ( 7.099999999999926814, 2.500000000000000000, -0.5928203230275541635 ) ) ;
#106321=CARTESIAN_POINT ( 'NONE',  ( 10.79999999999991367, 12.50000000000000000, -2.385244779468109755E-15 ) ) ;
#106322=EDGE_CURVE ( 'NONE', #122166, #59725, #88052, .T. ) ;
#106323=EDGE_LOOP ( 'NONE', ( #23493, #352 ) ) ;
#106324=DIRECTION ( 'NONE',  ( 0.000000000000000000, 0.000000000000000000, -1.000000000000000000 ) ) ;
#106325=CIRCLE ( 'NONE', #8115, 0.09999999999999982514 ) ;
#106326=ORIENTED_EDGE ( 'NONE', *, *, #128440, .F. ) ;
#106327=DIRECTION ( 'NONE',  ( 0.000000000000000000, 0.000000000000000000, 1.000000000000000000 ) ) ;
#106328=EDGE_CURVE ( 'NONE', #8654, #105036, #108951, .T. ) ;
#106329=ORIENTED_EDGE ( 'NONE', *, *, #103535, .T. ) ;
#106330=DIRECTION ( 'NONE',  ( 0.000000000000000000, 0.000000000000000000, 1.000000000000000000 ) ) ;
#106331=CARTESIAN_POINT ( 'NONE',  ( 9.999999999999948486, 2.500000000000000000, -4.330127018922201643 ) ) ;
#106332=AXIS2_PLACEMENT_3D ( 'NONE', #48018, #10016, #97742 ) ;
#106333=AXIS2_PLACEMENT_3D ( 'NONE', #24735, #27294, #65285 ) ;
#106334=ORIENTED_EDGE ( 'NONE', *, *, #72385, .T. ) ;
#106335=DIRECTION ( 'NONE',  ( -0.000000000000000000, 1.000000000000000000, -0.000000000000000000 ) ) ;
#106336=CARTESIAN_POINT ( 'NONE',  ( -8.550000000000009592, 2.500000000000000000, 6.941600689897073018 ) ) ;
#106337=EDGE_LOOP ( 'NONE', ( #18749, #64295 ) ) ;
#106338=EDGE_CURVE ( 'NONE', #83523, #85122, #10695, .T. ) ;
#106339=DIRECTION ( 'NONE',  ( 0.000000000000000000, 0.000000000000000000, -1.000000000000000000 ) ) ;
#106340=ORIENTED_EDGE ( 'NONE', *, *, #1380, .T. ) ;
#106341=ORIENTED_EDGE ( 'NONE', *, *, #53289, .F. ) ;
#106342=DIRECTION ( 'NONE',  ( -0.000000000000000000, -1.000000000000000000, -0.000000000000000000 ) ) ;
#106343=CARTESIAN_POINT ( 'NONE',  ( -0.6500000000000398792, 2.500000000000000000, -2.511473670974877948 ) ) ;
#106345=CARTESIAN_POINT ( 'NONE',  ( -7.900000000000011013, 12.50000000000000000, 4.265033745738159077 ) ) ;
#106346=AXIS2_PLACEMENT_3D ( 'NONE', #8110, #38234, #65738 ) ;
#106347=CONICAL_SURFACE ( 'NONE', #93827, 0.1000000000000002554, 0.003490658503988666988 ) ;
#106348=DIRECTION ( 'NONE',  ( -0.000000000000000000, -1.000000000000000000, -0.000000000000000000 ) ) ;
#106349=DIRECTION ( 'NONE',  ( -0.000000000000000000, -1.000000000000000000, -0.000000000000000000 ) ) ;
#106350=CIRCLE ( 'NONE', #91686, 0.1000000000000002554 ) ;
#106351=EDGE_LOOP ( 'NONE', ( #105296, #103060 ) ) ;
#106352=DIRECTION ( 'NONE',  ( 0.000000000000000000, -0.000000000000000000, 1.000000000000000000 ) ) ;
#106353=ORIENTED_EDGE ( 'NONE', *, *, #100305, .F. ) ;
#106354=VECTOR ( 'NONE', #110690, 1000.000000000000000 ) ;
#106355=AXIS2_PLACEMENT_3D ( 'NONE', #24142, #115068, #3218 ) ;
#106356=AXIS2_PLACEMENT_3D ( 'NONE', #64560, #63930, #103855 ) ;
#106357=DIRECTION ( 'NONE',  ( 0.000000000000000000, 1.000000000000000000, 0.000000000000000000 ) ) ;
#106358=CARTESIAN_POINT ( 'NONE',  ( -11.05000000000000249, 2.500000000000000000, -1.818653347947322141 ) ) ;
#106359=CARTESIAN_POINT ( 'NONE',  ( -8.350000000000012079, 2.500000000000000000, -2.857883832488653741 ) ) ;
#106360=CARTESIAN_POINT ( 'NONE',  ( -1.900000000000034106, 12.50000000000000000, 0.3464101615137735735 ) ) ;
#106361=ORIENTED_EDGE ( 'NONE', *, *, #12176, .T. ) ;
#106362=AXIS2_PLACEMENT_3D ( 'NONE', #109882, #42436, #21493 ) ;
#106363=AXIS2_PLACEMENT_3D ( 'NONE', #84959, #63396, #34602 ) ;
#106364=EDGE_CURVE ( 'NONE', #16861, #7100, #17346, .T. ) ;
#106365=DIRECTION ( 'NONE',  ( -0.000000000000000000, -1.000000000000000000, -0.000000000000000000 ) ) ;
#106366=CARTESIAN_POINT ( 'NONE',  ( 6.249999999999932498, 2.500000000000000000, 5.902370205355745192 ) ) ;
#106367=ORIENTED_EDGE ( 'NONE', *, *, #14908, .T. ) ;
#106368=CARTESIAN_POINT ( 'NONE',  ( 6.249999999999930722, 2.500000000000000000, 7.188010851410848723 ) ) ;
#106369=ADVANCED_FACE ( 'NONE', ( #59251 ), #67758, .T. ) ;
#106370=ORIENTED_EDGE ( 'NONE', *, *, #85536, .T. ) ;
#106371=ORIENTED_EDGE ( 'NONE', *, *, #57550, .T. ) ;
#106372=FACE_OUTER_BOUND ( 'NONE', #23530, .T. ) ;
#106373=AXIS2_PLACEMENT_3D ( 'NONE', #47675, #57491, #127518 ) ;
#106374=ORIENTED_EDGE ( 'NONE', *, *, #43108, .F. ) ;
#106375=DIRECTION ( 'NONE',  ( 0.000000000000000000, 0.000000000000000000, -1.000000000000000000 ) ) ;
#106376=DIRECTION ( 'NONE',  ( 0.000000000000000000, 0.000000000000000000, 1.000000000000000000 ) ) ;
#106377=CARTESIAN_POINT ( 'NONE',  ( -2.050000000000032685, 2.500000000000000000, -2.165063509461101710 ) ) ;
#106378=EDGE_LOOP ( 'NONE', ( #45598, #116137, #44003, #57716 ) ) ;
#106379=VECTOR ( 'NONE', #79795, 1000.000000000000000 ) ;
#106380=FACE_BOUND ( 'NONE', #52143, .T. ) ;
#106381=LINE ( 'NONE', #65146, #56258 ) ;
#106382=EDGE_LOOP ( 'NONE', ( #6959, #118229 ) ) ;
#106383=DIRECTION ( 'NONE',  ( 0.000000000000000000, 0.000000000000000000, -1.000000000000000000 ) ) ;
#106384=CARTESIAN_POINT ( 'NONE',  ( 9.599999999999914380, 2.500000000000000000, -4.330127018922201643 ) ) ;
#106385=AXIS2_PLACEMENT_3D ( 'NONE', #10696, #51318, #31040 ) ;
#106387=AXIS2_PLACEMENT_3D ( 'NONE', #78493, #107925, #69275 ) ;
#106388=AXIS2_PLACEMENT_3D ( 'NONE', #107105, #76382, #25995 ) ;
#106389=VERTEX_POINT ( 'NONE', #27185 ) ;
#106390=ORIENTED_EDGE ( 'NONE', *, *, #7591, .F. ) ;
#106391=DIRECTION ( 'NONE',  ( 0.000000000000000000, 1.000000000000000000, 0.000000000000000000 ) ) ;
#106392=CARTESIAN_POINT ( 'NONE',  ( -15.79999999999998117, 2.500000000000000000, 0.1000000000000000056 ) ) ;
#106393=DIRECTION ( 'NONE',  ( -4.274815082592931898E-19, -0.9999939076577903929, -0.003490651415223739937 ) ) ;
#106394=FACE_BOUND ( 'NONE', #2367, .T. ) ;
#106395=ORIENTED_EDGE ( 'NONE', *, *, #73947, .F. ) ;
#106397=VECTOR ( 'NONE', #12056, 1000.000000000000000 ) ;
#106398=CARTESIAN_POINT ( 'NONE',  ( 10.64999999999991331, 12.50000000000000000, 6.148780366869520897 ) ) ;
#106399=DIRECTION ( 'NONE',  ( -0.000000000000000000, 1.000000000000000000, -0.000000000000000000 ) ) ;
#106400=CIRCLE ( 'NONE', #100157, 0.06509327318403745899 ) ;
#106401=EDGE_CURVE ( 'NONE', #41959, #66137, #106847, .T. ) ;
#106402=FACE_OUTER_BOUND ( 'NONE', #80954, .T. ) ;
#106403=CARTESIAN_POINT ( 'NONE',  ( 1.049999999999954525, 2.500000000000000000, 1.918653347947321564 ) ) ;
#106404=CARTESIAN_POINT ( 'NONE',  ( 1.249999999999954259, 12.50000000000000000, -7.188010851410854052 ) ) ;
#106405=FACE_OUTER_BOUND ( 'NONE', #37810, .T. ) ;
#106406=DIRECTION ( 'NONE',  ( 0.000000000000000000, 0.000000000000000000, -1.000000000000000000 ) ) ;
#106407=AXIS2_PLACEMENT_3D ( 'NONE', #97112, #126581, #76837 ) ;
#106408=ADVANCED_FACE ( 'NONE', ( #8185 ), #76943, .T. ) ;
#106409=DIRECTION ( 'NONE',  ( -0.000000000000000000, -1.000000000000000000, -0.000000000000000000 ) ) ;
#106410=ORIENTED_EDGE ( 'NONE', *, *, #112538, .F. ) ;
#106412=EDGE_LOOP ( 'NONE', ( #119008, #35431, #111376, #51024 ) ) ;
#106413=ORIENTED_EDGE ( 'NONE', *, *, #124805, .T. ) ;
#106414=VERTEX_POINT ( 'NONE', #48130 ) ;
#106415=AXIS2_PLACEMENT_3D ( 'NONE', #16608, #87286, #87919 ) ;
#106416=CARTESIAN_POINT ( 'NONE',  ( -2.900000000000030109, 2.500000000000000000, -3.537306695894649966 ) ) ;
#106417=EDGE_CURVE ( 'NONE', #115797, #68417, #31657, .T. ) ;
#106418=FACE_OUTER_BOUND ( 'NONE', #31626, .T. ) ;
#106420=FACE_BOUND ( 'NONE', #51412, .T. ) ;
#106421=EDGE_CURVE ( 'NONE', #112463, #76648, #8639, .T. ) ;
#106422=DIRECTION ( 'NONE',  ( 0.000000000000000000, -0.000000000000000000, 1.000000000000000000 ) ) ;
#106423=AXIS2_PLACEMENT_3D ( 'NONE', #6819, #56577, #76248 ) ;
#106424=EDGE_CURVE ( 'NONE', #128284, #16041, #115235, .T. ) ;
#106425=DIRECTION ( 'NONE',  ( 0.000000000000000000, 1.000000000000000000, 0.000000000000000000 ) ) ;
#106426=CARTESIAN_POINT ( 'NONE',  ( 5.449999999999934452, 2.500000000000000000, 2.265063509461097357 ) ) ;
#106427=CARTESIAN_POINT ( 'NONE',  ( -0.6000000000000323963, 12.50000000000000000, 0.3464101615137759604 ) ) ;
#106428=EDGE_CURVE ( 'NONE', #32665, #72747, #81456, .T. ) ;
#106429=DIRECTION ( 'NONE',  ( -0.000000000000000000, -1.000000000000000000, -0.000000000000000000 ) ) ;
#106430=EDGE_LOOP ( 'NONE', ( #36407, #66748 ) ) ;
#106431=CIRCLE ( 'NONE', #102334, 0.06509327318403745899 ) ;
#106432=DIRECTION ( 'NONE',  ( 0.000000000000000000, 0.000000000000000000, -1.000000000000000000 ) ) ;
#106433=AXIS2_PLACEMENT_3D ( 'NONE', #43619, #103816, #42988 ) ;
#106434=VERTEX_POINT ( 'NONE', #82090 ) ;
#106435=ORIENTED_EDGE ( 'NONE', *, *, #65847, .F. ) ;
#106436=EDGE_LOOP ( 'NONE', ( #98926, #77316, #42, #27856 ) ) ;
#106437=CARTESIAN_POINT ( 'NONE',  ( -7.050000000000016698, 2.500000000000000000, -6.495190528383302464 ) ) ;
#106438=DIRECTION ( 'NONE',  ( 0.000000000000000000, 0.000000000000000000, -1.000000000000000000 ) ) ;
#106439=PLANE ( 'NONE',  #121999 ) ;
#106440=AXIS2_PLACEMENT_3D ( 'NONE', #30496, #62526, #82153 ) ;
#106441=ORIENTED_EDGE ( 'NONE', *, *, #69363, .F. ) ;
#106443=DIRECTION ( 'NONE',  ( 0.000000000000000000, 0.000000000000000000, 1.000000000000000000 ) ) ;
#106444=AXIS2_PLACEMENT_3D ( 'NONE', #26673, #39090, #126157 ) ;
#106445=DIRECTION ( 'NONE',  ( -0.000000000000000000, 1.000000000000000000, -0.000000000000000000 ) ) ;
#106446=AXIS2_PLACEMENT_3D ( 'NONE', #81606, #128810, #100593 ) ;
#106448=FACE_OUTER_BOUND ( 'NONE', #114952, .T. ) ;
#106449=CARTESIAN_POINT ( 'NONE',  ( 12.09999999999990550, 2.500000000000000000, -4.922947341949753586 ) ) ;
#106450=AXIS2_PLACEMENT_3D ( 'NONE', #95959, #36416, #48157 ) ;
#106451=DIRECTION ( 'NONE',  ( 0.000000000000000000, 1.000000000000000000, 0.000000000000000000 ) ) ;
#106452=VERTEX_POINT ( 'NONE', #10135 ) ;
#106453=PLANE ( 'NONE',  #106892 ) ;
#106454=AXIS2_PLACEMENT_3D ( 'NONE', #103923, #45011, #35827 ) ;
#106455=VECTOR ( 'NONE', #118285, 1000.000000000000000 ) ;
#106457=ORIENTED_EDGE ( 'NONE', *, *, #103796, .F. ) ;
#106458=FACE_OUTER_BOUND ( 'NONE', #27531, .T. ) ;
#106459=DIRECTION ( 'NONE',  ( 0.000000000000000000, 0.000000000000000000, -1.000000000000000000 ) ) ;
#106460=CARTESIAN_POINT ( 'NONE',  ( -8.750000000000010658, 12.50000000000000000, 2.857883832488649301 ) ) ;
#106461=ORIENTED_EDGE ( 'NONE', *, *, #24860, .T. ) ;
#106462=ORIENTED_EDGE ( 'NONE', *, *, #114965, .T. ) ;
#106463=EDGE_CURVE ( 'NONE', #92990, #77408, #52579, .T. ) ;
#106464=CARTESIAN_POINT ( 'NONE',  ( -7.499999999999980460, 12.50000000000000000, -4.330127018922201643 ) ) ;
#106465=DIRECTION ( 'NONE',  ( 0.000000000000000000, 0.000000000000000000, -1.000000000000000000 ) ) ;
#106466=DIRECTION ( 'NONE',  ( 0.000000000000000000, 1.000000000000000000, 0.000000000000000000 ) ) ;
#106467=EDGE_CURVE ( 'NONE', #36022, #61453, #54622, .T. ) ;
#106468=AXIS2_PLACEMENT_3D ( 'NONE', #46070, #66338, #106271 ) ;
#106470=ORIENTED_EDGE ( 'NONE', *, *, #40688, .F. ) ;
#106471=ADVANCED_FACE ( 'NONE', ( #52624 ), #41545, .T. ) ;
#106472=LINE ( 'NONE', #6954, #115018 ) ;
#106473=ADVANCED_FACE ( 'NONE', ( #89967 ), #12842, .T. ) ;
#106474=ADVANCED_FACE ( 'NONE', ( #21231 ), #123578, .T. ) ;
#106475=EDGE_LOOP ( 'NONE', ( #55182, #87534, #45639, #87455 ) ) ;
#106476=CARTESIAN_POINT ( 'NONE',  ( -6.900000000000019007, 2.500000000000000000, 0.3464101615137735735 ) ) ;
#106477=AXIS2_PLACEMENT_3D ( 'NONE', #114406, #115039, #64664 ) ;
#106478=VECTOR ( 'NONE', #83793, 1000.000000000000000 ) ;
#106479=PLANE ( 'NONE',  #84649 ) ;
#106480=ORIENTED_EDGE ( 'NONE', *, *, #114715, .T. ) ;
#106481=CARTESIAN_POINT ( 'NONE',  ( 1.449999999999950440, 12.50000000000000000, 6.148780366869520009 ) ) ;
#106482=EDGE_CURVE ( 'NONE', #935, #83109, #83869, .T. ) ;
#106483=FACE_OUTER_BOUND ( 'NONE', #121880, .T. ) ;
#106484=CARTESIAN_POINT ( 'NONE',  ( 8.349999999999923261, 12.50000000000000000, 2.792790559304612064 ) ) ;
#106485=CARTESIAN_POINT ( 'NONE',  ( -6.050000000000017586, 2.500000000000000000, 6.048780366869520364 ) ) ;
#106486=CIRCLE ( 'NONE', #37545, 0.06509327318403745899 ) ;
#106487=ORIENTED_EDGE ( 'NONE', *, *, #45714, .T. ) ;
#106488=AXIS2_PLACEMENT_3D ( 'NONE', #92817, #23401, #63343 ) ;
#106489=ADVANCED_FACE ( 'NONE', ( #72287 ), #96384, .T. ) ;
#106490=DIRECTION ( 'NONE',  ( 0.000000000000000000, 0.000000000000000000, 1.000000000000000000 ) ) ;
#106491=EDGE_CURVE ( 'NONE', #111625, #35458, #69289, .T. ) ;
#106492=DIRECTION ( 'NONE',  ( 0.000000000000000000, 0.000000000000000000, 1.000000000000000000 ) ) ;
#106493=ORIENTED_EDGE ( 'NONE', *, *, #104834, .F. ) ;
#106494=EDGE_LOOP ( 'NONE', ( #95850, #93147, #63008, #68090 ) ) ;
#106495=CARTESIAN_POINT ( 'NONE',  ( -0.6500000000000398792, 2.500000000000000000, -6.741600689897078169 ) ) ;
#106496=CARTESIAN_POINT ( 'NONE',  ( 10.39999999999991509, 2.500000000000000000, -0.6928203230275542523 ) ) ;
#106497=CARTESIAN_POINT ( 'NONE',  ( 10.84999999999990905, 2.500000000000000000, 2.957883832488649389 ) ) ;
#106498=DIRECTION ( 'NONE',  ( 0.000000000000000000, 0.000000000000000000, 1.000000000000000000 ) ) ;
#106499=CARTESIAN_POINT ( 'NONE',  ( -11.89999999999999680, 2.500000000000000000, -3.983716857408423628 ) ) ;
#106500=DIRECTION ( 'NONE',  ( 0.000000000000000000, 0.000000000000000000, 1.000000000000000000 ) ) ;
#106501=VECTOR ( 'NONE', #32201, 1000.000000000000000 ) ;
#106502=CARTESIAN_POINT ( 'NONE',  ( 18.00406199218825876, 1.510509990051560170, -4.944015969580407344 ) ) ;
#106503=DIRECTION ( 'NONE',  ( 0.000000000000000000, -0.000000000000000000, 1.000000000000000000 ) ) ;
#106504=DIRECTION ( 'NONE',  ( 0.000000000000000000, -0.000000000000000000, 1.000000000000000000 ) ) ;
#106505=CARTESIAN_POINT ( 'NONE',  ( 13.09999999999989839, 2.500000000000000000, 0.2464101615137735679 ) ) ;
#106506=ORIENTED_EDGE ( 'NONE', *, *, #52520, .T. ) ;
#106507=ORIENTED_EDGE ( 'NONE', *, *, #23526, .T. ) ;
#106508=AXIS2_PLACEMENT_3D ( 'NONE', #23075, #102909, #44012 ) ;
#106509=DIRECTION ( 'NONE',  ( -0.000000000000000000, -1.000000000000000000, -0.000000000000000000 ) ) ;
#106511=FACE_OUTER_BOUND ( 'NONE', #114033, .T. ) ;
#106513=DIRECTION ( 'NONE',  ( -0.000000000000000000, 1.000000000000000000, -0.000000000000000000 ) ) ;
#106514=VERTEX_POINT ( 'NONE', #121360 ) ;
#106515=DIRECTION ( 'NONE',  ( 0.000000000000000000, 0.000000000000000000, 1.000000000000000000 ) ) ;
#106516=LINE ( 'NONE', #96051, #111855 ) ;
#106517=DIRECTION ( 'NONE',  ( 0.000000000000000000, 0.000000000000000000, 1.000000000000000000 ) ) ;
#106518=ORIENTED_EDGE ( 'NONE', *, *, #119044, .T. ) ;
#106519=DIRECTION ( 'NONE',  ( 0.000000000000000000, -0.9999939076577903929, 0.003490651415223739937 ) ) ;
#106520=ORIENTED_EDGE ( 'NONE', *, *, #48272, .F. ) ;
#106521=EDGE_CURVE ( 'NONE', #55512, #72078, #79522, .T. ) ;
#106523=ORIENTED_EDGE ( 'NONE', *, *, #72879, .T. ) ;
#106524=ORIENTED_EDGE ( 'NONE', *, *, #80871, .T. ) ;
#106525=DIRECTION ( 'NONE',  ( 0.000000000000000000, -0.000000000000000000, 1.000000000000000000 ) ) ;
#106526=CIRCLE ( 'NONE', #108592, 0.06509327318403745899 ) ;
#106527=FACE_OUTER_BOUND ( 'NONE', #97520, .T. ) ;
#106529=FACE_OUTER_BOUND ( 'NONE', #3670, .T. ) ;
#106530=ORIENTED_EDGE ( 'NONE', *, *, #85308, .F. ) ;
#106531=CONICAL_SURFACE ( 'NONE', #96160, 0.1000000000000000472, 0.003490658503988666988 ) ;
#106532=AXIS2_PLACEMENT_3D ( 'NONE', #124758, #54086, #12214 ) ;
#106533=CARTESIAN_POINT ( 'NONE',  ( -9.200000000000006395, 12.50000000000000000, -2.385244779468109755E-15 ) ) ;
#106534=EDGE_LOOP ( 'NONE', ( #102765, #123248, #117425, #61664 ) ) ;
#106535=DIRECTION ( 'NONE',  ( -0.000000000000000000, -1.000000000000000000, -0.000000000000000000 ) ) ;
#106536=CARTESIAN_POINT ( 'NONE',  ( 13.39473262194572101, -2.500000000000000000, -7.044698189558706858 ) ) ;
#106537=VECTOR ( 'NONE', #1463, 1000.000000000000000 ) ;
#106538=CARTESIAN_POINT ( 'NONE',  ( -4.800000000000024691, 12.50000000000000000, 0.3464101615137735735 ) ) ;
#106539=CARTESIAN_POINT ( 'NONE',  ( -4.350000000000023626, 12.50000000000000000, -1.818653347947325916 ) ) ;
#106540=VERTEX_POINT ( 'NONE', #70338 ) ;
#106541=AXIS2_PLACEMENT_3D ( 'NONE', #29094, #11364, #39571 ) ;
#106542=AXIS2_PLACEMENT_3D ( 'NONE', #125063, #13150, #125688 ) ;
#106543=ORIENTED_EDGE ( 'NONE', *, *, #117971, .F. ) ;
#106544=ORIENTED_EDGE ( 'NONE', *, *, #116089, .F. ) ;
#106545=DIRECTION ( 'NONE',  ( 0.000000000000000000, -0.9999939076577903929, 0.003490651415223739937 ) ) ;
#106546=DIRECTION ( 'NONE',  ( 0.000000000000000000, 0.000000000000000000, 1.000000000000000000 ) ) ;
#106547=DIRECTION ( 'NONE',  ( -4.274815082592931898E-19, -0.9999939076577903929, -0.003490651415223739937 ) ) ;
#106548=FACE_BOUND ( 'NONE', #38523, .T. ) ;
#106550=FACE_OUTER_BOUND ( 'NONE', #30152, .T. ) ;
#106551=PLANE ( 'NONE',  #39287 ) ;
#106552=DIRECTION ( 'NONE',  ( 0.000000000000000000, 0.000000000000000000, 1.000000000000000000 ) ) ;
#106554=CARTESIAN_POINT ( 'NONE',  ( 0.6499999999999561684, 2.500000000000000000, 2.411473670974873862 ) ) ;
#106555=DIRECTION ( 'NONE',  ( -4.274815082592931898E-19, -0.9999939076577903929, -0.003490651415223739937 ) ) ;
#106556=AXIS2_PLACEMENT_3D ( 'NONE', #109598, #19930, #81430 ) ;
#106557=EDGE_CURVE ( 'NONE', #8586, #113064, #12684, .T. ) ;
#106558=DIRECTION ( 'NONE',  ( 0.000000000000000000, 0.000000000000000000, 1.000000000000000000 ) ) ;
#106559=ORIENTED_EDGE ( 'NONE', *, *, #87975, .T. ) ;
#106560=ORIENTED_EDGE ( 'NONE', *, *, #94154, .F. ) ;
#106561=ORIENTED_EDGE ( 'NONE', *, *, #116275, .F. ) ;
#106562=ORIENTED_EDGE ( 'NONE', *, *, #40519, .T. ) ;
#106563=ADVANCED_FACE ( 'NONE', ( #110261 ), #77607, .T. ) ;
#106564=CARTESIAN_POINT ( 'NONE',  ( 11.44999999999990870, 2.500000000000000000, -1.918653347947326004 ) ) ;
#106565=FACE_BOUND ( 'NONE', #50022, .T. ) ;
#106566=ADVANCED_FACE ( 'NONE', ( #10741 ), #21273, .T. ) ;
#106567=DIRECTION ( 'NONE',  ( 0.000000000000000000, 0.000000000000000000, 1.000000000000000000 ) ) ;
#106568=CIRCLE ( 'NONE', #48010, 0.06509327318403743123 ) ;
#106569=AXIS2_PLACEMENT_3D ( 'NONE', #30833, #88425, #29527 ) ;
#106570=DIRECTION ( 'NONE',  ( 0.000000000000000000, 1.000000000000000000, 0.000000000000000000 ) ) ;
#106571=ADVANCED_FACE ( 'NONE', ( #951 ), #39621, .T. ) ;
#106572=ADVANCED_FACE ( 'NONE', ( #51365 ), #91913, .T. ) ;
#106573=EDGE_LOOP ( 'NONE', ( #94618, #23331 ) ) ;
#106574=CARTESIAN_POINT ( 'NONE',  ( -11.05000000000000249, 2.500000000000000000, -1.718653347947322052 ) ) ;
#106575=EDGE_CURVE ( 'NONE', #77408, #92990, #23320, .T. ) ;
#106577=ADVANCED_FACE ( 'NONE', ( #13979 ), #52670, .T. ) ;
#106578=CONICAL_SURFACE ( 'NONE', #110692, 0.09999999999999982514, 0.003490658503988666988 ) ;
#106579=EDGE_LOOP ( 'NONE', ( #85976, #110372, #65180, #23254 ) ) ;
#106580=DIRECTION ( 'NONE',  ( -4.274815082592931898E-19, -0.9999939076577903929, -0.003490651415223739937 ) ) ;
#106581=CARTESIAN_POINT ( 'NONE',  ( 18.70618316909983392, 2.558637580971244496, -2.503050677946455416 ) ) ;
#106582=CIRCLE ( 'NONE', #125370, 0.06509327318403745899 ) ;
#106583=CIRCLE ( 'NONE', #123313, 0.1000000000000002554 ) ;
#106584=EDGE_LOOP ( 'NONE', ( #84081, #33839 ) ) ;
#106585=DIRECTION ( 'NONE',  ( 0.000000000000000000, 1.000000000000000000, 0.000000000000000000 ) ) ;
#106586=CARTESIAN_POINT ( 'NONE',  ( -3.950000000000024603, 2.500000000000000000, 1.718653347947321386 ) ) ;
#106587=CONICAL_SURFACE ( 'NONE', #43918, 0.09999999999999982514, 0.003490658503988666988 ) ;
#106588=ADVANCED_FACE ( 'NONE', ( #42846 ), #33011, .T. ) ;
#106589=CONICAL_SURFACE ( 'NONE', #117033, 0.09999999999999982514, 0.003490658503988666988 ) ;
#106590=VERTEX_POINT ( 'NONE', #53923 ) ;
#106591=DIRECTION ( 'NONE',  ( 0.000000000000000000, 1.000000000000000000, 0.000000000000000000 ) ) ;
#106592=DIRECTION ( 'NONE',  ( 0.000000000000000000, 1.000000000000000000, 0.000000000000000000 ) ) ;
#106593=VERTEX_POINT ( 'NONE', #54543 ) ;
#106594=CARTESIAN_POINT ( 'NONE',  ( -1.650000000000035660, 2.500000000000000000, 7.288010851410849256 ) ) ;
#106595=CIRCLE ( 'NONE', #94088, 0.06509327318403745899 ) ;
#106596=ORIENTED_EDGE ( 'NONE', *, *, #19105, .F. ) ;
#106597=VERTEX_POINT ( 'NONE', #84667 ) ;
#106598=CARTESIAN_POINT ( 'NONE',  ( 9.349999999999919709, 2.500000000000000000, -6.841600689897078702 ) ) ;
#106599=ORIENTED_EDGE ( 'NONE', *, *, #113890, .T. ) ;
#106600=LINE ( 'NONE', #25444, #95120 ) ;
#106601=DIRECTION ( 'NONE',  ( 0.000000000000000000, 1.000000000000000000, 0.000000000000000000 ) ) ;
#106602=ORIENTED_EDGE ( 'NONE', *, *, #99721, .F. ) ;
#106604=DIRECTION ( 'NONE',  ( 0.000000000000000000, 0.000000000000000000, 1.000000000000000000 ) ) ;
#106606=DIRECTION ( 'NONE',  ( 0.000000000000000000, 0.000000000000000000, -1.000000000000000000 ) ) ;
#106607=EDGE_CURVE ( 'NONE', #63275, #59954, #96473, .T. ) ;
#106608=FACE_OUTER_BOUND ( 'NONE', #110528, .T. ) ;
#106609=CARTESIAN_POINT ( 'NONE',  ( 17.50000000000011369, 2.262047038896492612, -3.993694673355268066 ) ) ;
#106610=VERTEX_POINT ( 'NONE', #74856 ) ;
#106611=ORIENTED_EDGE ( 'NONE', *, *, #44545, .T. ) ;
#106612=DIRECTION ( 'NONE',  ( 0.000000000000000000, 1.000000000000000000, 0.000000000000000000 ) ) ;
#106613=DIRECTION ( 'NONE',  ( 0.000000000000000000, 0.000000000000000000, 1.000000000000000000 ) ) ;
#106614=FACE_OUTER_BOUND ( 'NONE', #90040, .T. ) ;
#106615=ADVANCED_FACE ( 'NONE', ( #82757 ), #35581, .T. ) ;
#106616=ORIENTED_EDGE ( 'NONE', *, *, #17340, .T. ) ;
#106617=EDGE_LOOP ( 'NONE', ( #24091, #72589 ) ) ;
#106618=EDGE_LOOP ( 'NONE', ( #102508, #97277, #126841, #54607 ) ) ;
#106619=EDGE_CURVE ( 'NONE', #61864, #104101, #14614, .T. ) ;
#106621=DIRECTION ( 'NONE',  ( 0.000000000000000000, 0.000000000000000000, -1.000000000000000000 ) ) ;
#106622=ADVANCED_FACE ( 'NONE', ( #64379 ), #19202, .T. ) ;
#106623=DIRECTION ( 'NONE',  ( 0.000000000000000000, 0.000000000000000000, -1.000000000000000000 ) ) ;
#106624=DIRECTION ( 'NONE',  ( 0.000000000000000000, 1.000000000000000000, 0.000000000000000000 ) ) ;
#106625=ADVANCED_FACE ( 'NONE', ( #93848 ), #114765, .T. ) ;
#106627=VECTOR ( 'NONE', #63714, 1000.000000000000000 ) ;
#106628=AXIS2_PLACEMENT_3D ( 'NONE', #42336, #75017, #12839 ) ;
#106629=DIRECTION ( 'NONE',  ( -0.000000000000000000, -1.000000000000000000, -0.000000000000000000 ) ) ;
#106630=DIRECTION ( 'NONE',  ( -4.274815082592931898E-19, -0.9999939076577903929, -0.003490651415223739937 ) ) ;
#106631=DIRECTION ( 'NONE',  ( 0.000000000000000000, -0.9999939076577903929, 0.003490651415223739937 ) ) ;
#106632=CARTESIAN_POINT ( 'NONE',  ( 6.249999999999928946, 2.500000000000000000, 2.857883832488649301 ) ) ;
#106633=CARTESIAN_POINT ( 'NONE',  ( 9.149999999999918643, 2.500000000000000000, 2.065063509461097624 ) ) ;
#106634=EDGE_CURVE ( 'NONE', #90933, #112226, #119464, .T. ) ;
#106635=EDGE_CURVE ( 'NONE', #39561, #65655, #63135, .T. ) ;
#106636=CARTESIAN_POINT ( 'NONE',  ( -2.300000000000032685, 2.500000000000000000, -4.776537180435978414 ) ) ;
#106637=ADVANCED_FACE ( 'NONE', ( #74209 ), #38002, .T. ) ;
#106638=AXIS2_PLACEMENT_3D ( 'NONE', #95735, #17123, #47282 ) ;
#106639=EDGE_CURVE ( 'NONE', #92080, #46749, #81901, .T. ) ;
#106640=EDGE_LOOP ( 'NONE', ( #13552, #46099 ) ) ;
#106641=ADVANCED_FACE ( 'NONE', ( #115385 ), #85306, .T. ) ;
#106643=EDGE_LOOP ( 'NONE', ( #93231, #75135 ) ) ;
#106644=ORIENTED_EDGE ( 'NONE', *, *, #54149, .T. ) ;
#106645=CARTESIAN_POINT ( 'NONE',  ( -9.350000000000004974, 12.50000000000000000, 6.148780366869520897 ) ) ;
#106646=DIRECTION ( 'NONE',  ( 0.000000000000000000, -0.000000000000000000, 1.000000000000000000 ) ) ;
#106647=CARTESIAN_POINT ( 'NONE',  ( 0.8499999999999536815, 12.50000000000000000, 5.737276932171707422 ) ) ;
#106648=EDGE_CURVE ( 'NONE', #96223, #75562, #12944, .T. ) ;
#106649=FACE_OUTER_BOUND ( 'NONE', #6624, .T. ) ;
#106650=DIRECTION ( 'NONE',  ( -0.000000000000000000, -1.000000000000000000, -0.000000000000000000 ) ) ;
#106651=CARTESIAN_POINT ( 'NONE',  ( -11.05000000000000071, 2.500000000000000000, -6.841600689897075149 ) ) ;
#106652=DIRECTION ( 'NONE',  ( -0.000000000000000000, 1.000000000000000000, -0.000000000000000000 ) ) ;
#106653=EDGE_LOOP ( 'NONE', ( #6850, #14700 ) ) ;
#106654=DIRECTION ( 'NONE',  ( -0.000000000000000000, 1.000000000000000000, -0.000000000000000000 ) ) ;
#106655=DIRECTION ( 'NONE',  ( -4.274815082592931898E-19, -0.9999939076577903929, -0.003490651415223739937 ) ) ;
#106656=VERTEX_POINT ( 'NONE', #65662 ) ;
#106657=CIRCLE ( 'NONE', #8440, 0.1000000000000002554 ) ;
#106658=EDGE_LOOP ( 'NONE', ( #83, #14985, #73656, #121410 ) ) ;
#106659=ORIENTED_EDGE ( 'NONE', *, *, #109368, .F. ) ;
#106660=ORIENTED_EDGE ( 'NONE', *, *, #59997, .T. ) ;
#106661=VERTEX_POINT ( 'NONE', #105609 ) ;
#106662=CARTESIAN_POINT ( 'NONE',  ( 1.049999999999954525, 2.500000000000000000, -2.611473670974877592 ) ) ;
#106663=CARTESIAN_POINT ( 'NONE',  ( -11.25000000000000000, 12.50000000000000000, -2.857883832488649745 ) ) ;
#106664=VECTOR ( 'NONE', #120388, 1000.000000000000000 ) ;
#106665=ORIENTED_EDGE ( 'NONE', *, *, #85031, .F. ) ;
#106666=CARTESIAN_POINT ( 'NONE',  ( -10.00000000000000355, 12.50000000000000000, -0.6928203230275541413 ) ) ;
#106667=CARTESIAN_POINT ( 'NONE',  ( -6.250000000000021316, 2.500000000000000000, -5.902370205355750521 ) ) ;
#106668=FACE_OUTER_BOUND ( 'NONE', #106494, .T. ) ;
#106669=ORIENTED_EDGE ( 'NONE', *, *, #75127, .F. ) ;
#106670=CARTESIAN_POINT ( 'NONE',  ( 12.49999999999993960, 2.500000000000000000, -4.430127018922202176 ) ) ;
#106672=CARTESIAN_POINT ( 'NONE',  ( -8.350000000000008527, 2.500000000000000000, 7.088010851410848190 ) ) ;
#106673=VECTOR ( 'NONE', #64183, 1000.000000000000000 ) ;
#106674=ORIENTED_EDGE ( 'NONE', *, *, #89787, .F. ) ;
#106675=AXIS2_PLACEMENT_3D ( 'NONE', #98981, #13647, #108785 ) ;
#106676=EDGE_CURVE ( 'NONE', #37339, #89951, #104885, .T. ) ;
#106677=VERTEX_POINT ( 'NONE', #112848 ) ;
#106678=ORIENTED_EDGE ( 'NONE', *, *, #128287, .F. ) ;
#106679=DIRECTION ( 'NONE',  ( 0.000000000000000000, 1.000000000000000000, 0.000000000000000000 ) ) ;
#106680=VECTOR ( 'NONE', #113149, 1000.000000000000000 ) ;
#106681=DIRECTION ( 'NONE',  ( 0.000000000000000000, 0.000000000000000000, 1.000000000000000000 ) ) ;
#106682=CIRCLE ( 'NONE', #75381, 0.1000000000000002554 ) ;
#106683=ORIENTED_EDGE ( 'NONE', *, *, #35200, .T. ) ;
#106684=DIRECTION ( 'NONE',  ( -0.000000000000000000, -1.000000000000000000, -0.000000000000000000 ) ) ;
#106685=CARTESIAN_POINT ( 'NONE',  ( -8.550000000000014921, 12.50000000000000000, -6.148780366869520897 ) ) ;
#106686=ADVANCED_FACE ( 'NONE', ( #83392 ), #73499, .T. ) ;
#106687=DIRECTION ( 'NONE',  ( 0.000000000000000000, 0.000000000000000000, 1.000000000000000000 ) ) ;
#106688=CARTESIAN_POINT ( 'NONE',  ( -9.150000000000009237, 12.50000000000000000, -2.857883832488653741 ) ) ;
#106689=ORIENTED_EDGE ( 'NONE', *, *, #40403, .F. ) ;
#106690=FACE_OUTER_BOUND ( 'NONE', #123178, .T. ) ;
#106691=ORIENTED_EDGE ( 'NONE', *, *, #78854, .F. ) ;
#106692=ORIENTED_EDGE ( 'NONE', *, *, #110405, .T. ) ;
#106693=EDGE_LOOP ( 'NONE', ( #94138, #10275, #66608, #4407 ) ) ;
#106694=DIRECTION ( 'NONE',  ( 0.000000000000000000, 0.000000000000000000, 1.000000000000000000 ) ) ;
#106695=FACE_BOUND ( 'NONE', #16435, .T. ) ;
#106696=DIRECTION ( 'NONE',  ( 0.000000000000000000, 0.000000000000000000, 1.000000000000000000 ) ) ;
#106697=DIRECTION ( 'NONE',  ( 0.000000000000000000, 0.000000000000000000, 1.000000000000000000 ) ) ;
#106698=DIRECTION ( 'NONE',  ( -0.000000000000000000, 1.000000000000000000, -0.000000000000000000 ) ) ;
#106699=AXIS2_PLACEMENT_3D ( 'NONE', #17428, #18736, #7617 ) ;
#106700=VERTEX_POINT ( 'NONE', #107534 ) ;
#106701=CARTESIAN_POINT ( 'NONE',  ( 6.849999999999930367, 2.500000000000000000, -6.048780366869526581 ) ) ;
#106702=AXIS2_PLACEMENT_3D ( 'NONE', #12275, #123520, #101326 ) ;
#106704=CARTESIAN_POINT ( 'NONE',  ( -9.150000000000005684, 2.500000000000000000, 6.495190528383297135 ) ) ;
#106705=CARTESIAN_POINT ( 'NONE',  ( -14.14999999999998792, 2.500000000000000000, 2.857883832488652853 ) ) ;
#106706=ORIENTED_EDGE ( 'NONE', *, *, #95407, .F. ) ;
#106707=CARTESIAN_POINT ( 'NONE',  ( 14.59999999999989484, 2.500000000000000000, 0.5928203230275495006 ) ) ;
#106708=ADVANCED_FACE ( 'NONE', ( #128481 ), #63049, .T. ) ;
#106709=AXIS2_PLACEMENT_3D ( 'NONE', #51335, #80128, #91881 ) ;
#106710=DIRECTION ( 'NONE',  ( -0.000000000000000000, 1.000000000000000000, -0.000000000000000000 ) ) ;
#106711=ORIENTED_EDGE ( 'NONE', *, *, #76312, .T. ) ;
#106712=CARTESIAN_POINT ( 'NONE',  ( -7.100000000000013856, 2.500000000000000000, 4.922947341949748257 ) ) ;
#106713=DIRECTION ( 'NONE',  ( 0.000000000000000000, 0.000000000000000000, -1.000000000000000000 ) ) ;
#106714=FACE_BOUND ( 'NONE', #118609, .T. ) ;
#106715=ADVANCED_FACE ( 'NONE', ( #28337 ), #17028, .T. ) ;
#106717=EDGE_LOOP ( 'NONE', ( #91693, #7400, #90967, #92626 ) ) ;
#106718=FACE_OUTER_BOUND ( 'NONE', #63669, .T. ) ;
#106719=ADVANCED_FACE ( 'NONE', ( #125868 ), #117985, .T. ) ;
#106720=VERTEX_POINT ( 'NONE', #8029 ) ;
#106721=EDGE_CURVE ( 'NONE', #54523, #82469, #329, .T. ) ;
#106722=EDGE_LOOP ( 'NONE', ( #13899, #95598, #53588, #48680 ) ) ;
#106723=DIRECTION ( 'NONE',  ( -4.274815082592931898E-19, -0.9999939076577903929, -0.003490651415223739937 ) ) ;
#106724=ADVANCED_FACE ( 'NONE', ( #68243 ), #67205, .T. ) ;
#106725=EDGE_CURVE ( 'NONE', #30920, #55758, #48468, .T. ) ;
#106727=EDGE_CURVE ( 'NONE', #19758, #69648, #36227, .T. ) ;
#106728=VERTEX_POINT ( 'NONE', #127190 ) ;
#106729=CARTESIAN_POINT ( 'NONE',  ( -8.150000000000012790, 12.50000000000000000, 2.446380397790835826 ) ) ;
#106730=DIRECTION ( 'NONE',  ( -0.000000000000000000, -1.000000000000000000, -0.000000000000000000 ) ) ;
#106731=DIRECTION ( 'NONE',  ( -0.000000000000000000, -1.000000000000000000, -0.000000000000000000 ) ) ;
#106733=EDGE_CURVE ( 'NONE', #66584, #41461, #75638, .T. ) ;
#106735=AXIS2_PLACEMENT_3D ( 'NONE', #78006, #117924, #29553 ) ;
#106736=ADVANCED_FACE ( 'NONE', ( #19124 ), #26409, .T. ) ;
#106737=CIRCLE ( 'NONE', #18910, 0.1000000000000002554 ) ;
#106738=VERTEX_POINT ( 'NONE', #46681 ) ;
#106739=DIRECTION ( 'NONE',  ( -0.000000000000000000, 1.000000000000000000, -0.000000000000000000 ) ) ;
#106740=DIRECTION ( 'NONE',  ( 0.000000000000000000, 0.000000000000000000, 1.000000000000000000 ) ) ;
#106741=CARTESIAN_POINT ( 'NONE',  ( 0.8499999999999557909, 12.50000000000000000, -7.188010851410854052 ) ) ;
#106742=DIRECTION ( 'NONE',  ( 0.000000000000000000, 0.000000000000000000, 1.000000000000000000 ) ) ;
#106743=ORIENTED_EDGE ( 'NONE', *, *, #73398, .T. ) ;
#106744=CARTESIAN_POINT ( 'NONE',  ( -10.85000000000000142, 2.500000000000000000, -7.288010851410851032 ) ) ;
#106745=VERTEX_POINT ( 'NONE', #8658 ) ;
#106746=DIRECTION ( 'NONE',  ( 0.000000000000000000, 0.000000000000000000, -1.000000000000000000 ) ) ;
#106747=CARTESIAN_POINT ( 'NONE',  ( 13.74999999999989519, 2.500000000000000000, -2.857883832488653741 ) ) ;
#106748=AXIS2_PLACEMENT_3D ( 'NONE', #82246, #71778, #52138 ) ;
#106749=ORIENTED_EDGE ( 'NONE', *, *, #93165, .T. ) ;
#106750=DIRECTION ( 'NONE',  ( 0.000000000000000000, -0.9999939076577903929, 0.003490651415223739937 ) ) ;
#106751=DIRECTION ( 'NONE',  ( 0.000000000000000000, 0.000000000000000000, -1.000000000000000000 ) ) ;
#106752=CARTESIAN_POINT ( 'NONE',  ( -10.65000000000000391, 2.500000000000000000, -2.511473670974873951 ) ) ;
#106753=DIRECTION ( 'NONE',  ( 0.000000000000000000, 1.000000000000000000, 0.000000000000000000 ) ) ;
#106754=EDGE_LOOP ( 'NONE', ( #48935, #109044, #16678, #78555 ) ) ;
#106755=DIRECTION ( 'NONE',  ( 0.000000000000000000, 1.000000000000000000, 0.000000000000000000 ) ) ;
#106756=CARTESIAN_POINT ( 'NONE',  ( -5.650000000000023448, 2.500000000000000000, -2.411473670974877859 ) ) ;
#106757=DIRECTION ( 'NONE',  ( -0.000000000000000000, -1.000000000000000000, -0.000000000000000000 ) ) ;
#106758=DIRECTION ( 'NONE',  ( -0.000000000000000000, -1.000000000000000000, -0.000000000000000000 ) ) ;
#106759=DIRECTION ( 'NONE',  ( -4.274815082592931898E-19, -0.9999939076577903929, -0.003490651415223739937 ) ) ;
#106760=CIRCLE ( 'NONE', #90032, 0.1000000000000000472 ) ;
#106761=ORIENTED_EDGE ( 'NONE', *, *, #10260, .F. ) ;
#106762=AXIS2_PLACEMENT_3D ( 'NONE', #23979, #36388, #63249 ) ;
#106763=EDGE_LOOP ( 'NONE', ( #37008, #7690, #49115, #61489 ) ) ;
#106765=VERTEX_POINT ( 'NONE', #106244 ) ;
#106766=CARTESIAN_POINT ( 'NONE',  ( 11.89999999999990798, 12.50000000000000000, 4.611443907251934426 ) ) ;
#106767=ORIENTED_EDGE ( 'NONE', *, *, #41319, .F. ) ;
#106768=ORIENTED_EDGE ( 'NONE', *, *, #5764, .F. ) ;
#106769=EDGE_LOOP ( 'NONE', ( #102446, #20977, #10154, #65635 ) ) ;
#106770=DIRECTION ( 'NONE',  ( 0.000000000000000000, 0.000000000000000000, 1.000000000000000000 ) ) ;
#106771=AXIS2_PLACEMENT_3D ( 'NONE', #32692, #72596, #22864 ) ;
#106772=CARTESIAN_POINT ( 'NONE',  ( -15.59999999999998010, 2.500000000000000000, 0.3464101615137759604 ) ) ;
#106773=DIRECTION ( 'NONE',  ( 0.000000000000000000, 0.000000000000000000, -1.000000000000000000 ) ) ;
#106774=CARTESIAN_POINT ( 'NONE',  ( 10.59999999999991260, 2.500000000000000000, 0.3464101615137735735 ) ) ;
#106775=AXIS2_PLACEMENT_3D ( 'NONE', #89984, #80181, #118808 ) ;
#106776=DIRECTION ( 'NONE',  ( -0.000000000000000000, 1.000000000000000000, -0.000000000000000000 ) ) ;
#106777=DIRECTION ( 'NONE',  ( 0.000000000000000000, 1.000000000000000000, 0.000000000000000000 ) ) ;
#106778=EDGE_LOOP ( 'NONE', ( #109670, #112047, #39416, #94698 ) ) ;
#106779=EDGE_CURVE ( 'NONE', #82663, #115112, #86097, .T. ) ;
#106780=FACE_OUTER_BOUND ( 'NONE', #33226, .T. ) ;
#106781=ORIENTED_EDGE ( 'NONE', *, *, #98807, .T. ) ;
#106783=ORIENTED_EDGE ( 'NONE', *, *, #122220, .T. ) ;
#106784=EDGE_LOOP ( 'NONE', ( #77069, #53482 ) ) ;
#106785=ORIENTED_EDGE ( 'NONE', *, *, #28316, .F. ) ;
#106786=EDGE_CURVE ( 'NONE', #120673, #127817, #10783, .T. ) ;
#106787=CARTESIAN_POINT ( 'NONE',  ( 2.899999999999944844, 2.500000000000000000, 3.637306695894644726 ) ) ;
#106788=ORIENTED_EDGE ( 'NONE', *, *, #40833, .T. ) ;
#106789=EDGE_LOOP ( 'NONE', ( #28073, #101649, #87446, #12412 ) ) ;
#106790=EDGE_CURVE ( 'NONE', #14841, #896, #127811, .T. ) ;
#106791=CARTESIAN_POINT ( 'NONE',  ( -9.600000000000006750, 2.500000000000000000, 3.737306695894644371 ) ) ;
#106792=DIRECTION ( 'NONE',  ( 0.000000000000000000, 0.000000000000000000, -1.000000000000000000 ) ) ;
#106793=CARTESIAN_POINT ( 'NONE',  ( 13.14999999999989733, 12.50000000000000000, -1.818653347947325916 ) ) ;
#106794=DIRECTION ( 'NONE',  ( 0.000000000000000000, 1.000000000000000000, 0.000000000000000000 ) ) ;
#106795=CIRCLE ( 'NONE', #90070, 0.1000000000000002554 ) ;
#106796=DIRECTION ( 'NONE',  ( 0.000000000000000000, 0.000000000000000000, -1.000000000000000000 ) ) ;
#106797=ORIENTED_EDGE ( 'NONE', *, *, #69950, .T. ) ;
#106798=CONICAL_SURFACE ( 'NONE', #50371, 0.09999999999999982514, 0.003490658503988666988 ) ;
#106799=VECTOR ( 'NONE', #4232, 1000.000000000000000 ) ;
#106800=DIRECTION ( 'NONE',  ( -0.000000000000000000, -1.000000000000000000, -0.000000000000000000 ) ) ;
#106801=ORIENTED_EDGE ( 'NONE', *, *, #5386, .F. ) ;
#106802=DIRECTION ( 'NONE',  ( -4.274815082592931898E-19, -0.9999939076577903929, -0.003490651415223739937 ) ) ;
#106803=VECTOR ( 'NONE', #78702, 1000.000000000000000 ) ;
#106804=ORIENTED_EDGE ( 'NONE', *, *, #12466, .F. ) ;
#106805=CARTESIAN_POINT ( 'NONE',  ( -13.74999999999998934, 12.50000000000000000, -1.472243186433547901 ) ) ;
#106806=ORIENTED_EDGE ( 'NONE', *, *, #51906, .T. ) ;
#106807=ADVANCED_FACE ( 'NONE', ( #97703 ), #54710, .T. ) ;
#106808=EDGE_LOOP ( 'NONE', ( #87038, #10338, #91415, #88651 ) ) ;
#106809=DIRECTION ( 'NONE',  ( -0.000000000000000000, -1.000000000000000000, -0.000000000000000000 ) ) ;
#106810=DIRECTION ( 'NONE',  ( -0.000000000000000000, -1.000000000000000000, -0.000000000000000000 ) ) ;
#106811=CARTESIAN_POINT ( 'NONE',  ( 0.6499999999999543920, 12.50000000000000000, 6.148780366869520897 ) ) ;
#106812=DIRECTION ( 'NONE',  ( 0.000000000000000000, 1.000000000000000000, 0.000000000000000000 ) ) ;
#106813=DIRECTION ( 'NONE',  ( 0.000000000000000000, 1.000000000000000000, 0.000000000000000000 ) ) ;
#106814=ORIENTED_EDGE ( 'NONE', *, *, #5055, .F. ) ;
#106815=DIRECTION ( 'NONE',  ( 0.000000000000000000, 1.000000000000000000, 0.000000000000000000 ) ) ;
#106816=DIRECTION ( 'NONE',  ( 0.000000000000000000, -0.9999939076577903929, 0.003490651415223739937 ) ) ;
#106817=DIRECTION ( 'NONE',  ( -0.000000000000000000, 1.000000000000000000, -0.000000000000000000 ) ) ;
#106818=CARTESIAN_POINT ( 'NONE',  ( 11.89999999999990798, 12.50000000000000000, 4.048810130592458201 ) ) ;
#106819=CARTESIAN_POINT ( 'NONE',  ( 12.89999999999990266, 12.50000000000000000, -3.572213422710612374 ) ) ;
#106821=CIRCLE ( 'NONE', #31630, 0.1000000000000002554 ) ;
#106822=ADVANCED_FACE ( 'NONE', ( #6088 ), #4608, .T. ) ;
#106823=ORIENTED_EDGE ( 'NONE', *, *, #43422, .F. ) ;
#106824=DIRECTION ( 'NONE',  ( 0.000000000000000000, 0.000000000000000000, -1.000000000000000000 ) ) ;
#106825=ORIENTED_EDGE ( 'NONE', *, *, #75285, .F. ) ;
#106826=CARTESIAN_POINT ( 'NONE',  ( 4.799999999999935874, 2.500000000000000000, 3.983716857408420964 ) ) ;
#106827=CIRCLE ( 'NONE', #50399, 0.06509327318403745899 ) ;
#106828=CARTESIAN_POINT ( 'NONE',  ( -11.05000000000000071, 2.500000000000000000, -2.511473670974873951 ) ) ;
#106829=AXIS2_PLACEMENT_3D ( 'NONE', #28570, #108406, #58677 ) ;
#106830=VERTEX_POINT ( 'NONE', #81299 ) ;
#106832=PLANE ( 'NONE',  #32766 ) ;
#106833=DIRECTION ( 'NONE',  ( 0.000000000000000000, 1.000000000000000000, 0.000000000000000000 ) ) ;
#106835=FACE_OUTER_BOUND ( 'NONE', #62620, .T. ) ;
#106836=CARTESIAN_POINT ( 'NONE',  ( -9.550000000000002487, 12.50000000000000000, 6.495190528383297135 ) ) ;
#106837=EDGE_LOOP ( 'NONE', ( #15032, #78831, #18042, #99382 ) ) ;
#106838=VECTOR ( 'NONE', #52555, 1000.000000000000000 ) ;
#106839=CONICAL_SURFACE ( 'NONE', #85909, 0.1000000000000000472, 0.003490658503988666988 ) ;
#106840=CARTESIAN_POINT ( 'NONE',  ( 3.749999999999940492, 2.500000000000000000, 5.802370205355744659 ) ) ;
#106841=LINE ( 'NONE', #107505, #12155 ) ;
#106842=EDGE_LOOP ( 'NONE', ( #96083, #16361, #42087, #92142 ) ) ;
#106843=CARTESIAN_POINT ( 'NONE',  ( 13.34999999999990017, 2.500000000000000000, 2.165063509461097713 ) ) ;
#106844=FACE_OUTER_BOUND ( 'NONE', #64477, .T. ) ;
#106845=CARTESIAN_POINT ( 'NONE',  ( -5.450000000000019718, 12.50000000000000000, 2.165063509461097713 ) ) ;
#106846=CIRCLE ( 'NONE', #100594, 0.1000000000000002554 ) ;
#106847=CIRCLE ( 'NONE', #35859, 0.1000000000000002554 ) ;
#106848=EDGE_LOOP ( 'NONE', ( #123699, #50285 ) ) ;
#106849=DIRECTION ( 'NONE',  ( 0.000000000000000000, 1.000000000000000000, 0.000000000000000000 ) ) ;
#106850=VERTEX_POINT ( 'NONE', #121212 ) ;
#106852=FACE_OUTER_BOUND ( 'NONE', #120645, .T. ) ;
#106853=AXIS2_PLACEMENT_3D ( 'NONE', #64535, #23981, #105760 ) ;
#106854=CARTESIAN_POINT ( 'NONE',  ( -0.4500000000000397571, 2.500000000000000000, -6.395190528383301931 ) ) ;
#106855=EDGE_LOOP ( 'NONE', ( #43138, #23161, #66148, #85310 ) ) ;
#106856=DIRECTION ( 'NONE',  ( 0.000000000000000000, 0.000000000000000000, 1.000000000000000000 ) ) ;
#106857=ADVANCED_FACE ( 'NONE', ( #100919 ), #63225, .T. ) ;
#106858=CARTESIAN_POINT ( 'NONE',  ( -3.950000000000026379, 2.500000000000000000, -1.918653347947326004 ) ) ;
#106859=CONICAL_SURFACE ( 'NONE', #67048, 0.1000000000000000472, 0.003490658503988666988 ) ;
#106860=CONICAL_SURFACE ( 'NONE', #92199, 0.09999999999999982514, 0.003490658503988666988 ) ;
#106861=ORIENTED_EDGE ( 'NONE', *, *, #64482, .T. ) ;
#106862=FACE_OUTER_BOUND ( 'NONE', #79293, .T. ) ;
#106863=VERTEX_POINT ( 'NONE', #89182 ) ;
#106864=DIRECTION ( 'NONE',  ( 0.000000000000000000, -0.000000000000000000, 1.000000000000000000 ) ) ;
#106865=EDGE_CURVE ( 'NONE', #84166, #99722, #2563, .T. ) ;
#106866=ORIENTED_EDGE ( 'NONE', *, *, #102342, .T. ) ;
#106867=CARTESIAN_POINT ( 'NONE',  ( 3.549999999999942979, 2.500000000000000000, 1.818653347947321475 ) ) ;
#106868=DIRECTION ( 'NONE',  ( 0.000000000000000000, -0.9999939076577903929, 0.003490651415223739937 ) ) ;
#106869=EDGE_CURVE ( 'NONE', #47559, #104184, #30921, .T. ) ;
#106870=ORIENTED_EDGE ( 'NONE', *, *, #97547, .T. ) ;
#106873=EDGE_CURVE ( 'NONE', #64820, #15926, #71541, .T. ) ;
#106874=EDGE_CURVE ( 'NONE', #57584, #76809, #54808, .T. ) ;
#106875=CARTESIAN_POINT ( 'NONE',  ( 0.1999999999999576006, 2.500000000000000000, -4.776537180435978414 ) ) ;
#106876=CARTESIAN_POINT ( 'NONE',  ( 8.949999999999919353, 2.500000000000000000, 2.411473670974873862 ) ) ;
#106877=VERTEX_POINT ( 'NONE', #99652 ) ;
#106878=CARTESIAN_POINT ( 'NONE',  ( -13.34999999999999076, 12.50000000000000000, -2.792790559304614284 ) ) ;
#106879=CARTESIAN_POINT ( 'NONE',  ( 8.349999999999919709, 12.50000000000000000, -2.099970236277064473 ) ) ;
#106880=ADVANCED_FACE ( 'NONE', ( #9976 ), #59032, .T. ) ;
#106881=DIRECTION ( 'NONE',  ( -0.000000000000000000, -1.000000000000000000, -0.000000000000000000 ) ) ;
#106882=DIRECTION ( 'NONE',  ( -0.000000000000000000, -1.000000000000000000, -0.000000000000000000 ) ) ;
#106883=CIRCLE ( 'NONE', #16971, 0.09999999999999982514 ) ;
#106884=AXIS2_PLACEMENT_3D ( 'NONE', #49359, #129215, #39549 ) ;
#106885=EDGE_CURVE ( 'NONE', #126604, #96497, #41388, .T. ) ;
#106886=DIRECTION ( 'NONE',  ( -4.274815082592931898E-19, -0.9999939076577903929, -0.003490651415223739937 ) ) ;
#106887=CARTESIAN_POINT ( 'NONE',  ( -5.850000000000018296, 12.50000000000000000, 2.922977105672686982 ) ) ;
#106888=EDGE_CURVE ( 'NONE', #16778, #67980, #8830, .T. ) ;
#106889=EDGE_CURVE ( 'NONE', #62695, #108184, #104972, .T. ) ;
#106890=EDGE_CURVE ( 'NONE', #90081, #121723, #15071, .T. ) ;
#106891=ORIENTED_EDGE ( 'NONE', *, *, #67033, .T. ) ;
#106892=AXIS2_PLACEMENT_3D ( 'NONE', #65226, #114336, #123506 ) ;
#106893=ORIENTED_EDGE ( 'NONE', *, *, #76024, .F. ) ;
#106894=ORIENTED_EDGE ( 'NONE', *, *, #47482, .T. ) ;
#106895=VERTEX_POINT ( 'NONE', #60389 ) ;
#106896=FACE_OUTER_BOUND ( 'NONE', #59489, .T. ) ;
#106897=DIRECTION ( 'NONE',  ( 0.000000000000000000, 0.000000000000000000, 1.000000000000000000 ) ) ;
#106898=AXIS2_PLACEMENT_3D ( 'NONE', #127253, #99725, #77489 ) ;
#106899=DIRECTION ( 'NONE',  ( -4.274815082592931898E-19, -0.9999939076577903929, -0.003490651415223739937 ) ) ;
#106900=ORIENTED_EDGE ( 'NONE', *, *, #19506, .F. ) ;
#106901=FACE_BOUND ( 'NONE', #3099, .T. ) ;
#106902=EDGE_CURVE ( 'NONE', #107807, #28723, #84055, .T. ) ;
#106903=CARTESIAN_POINT ( 'NONE',  ( -8.950000000000009948, 2.500000000000000000, 2.511473670974873507 ) ) ;
#106904=CARTESIAN_POINT ( 'NONE',  ( -12.69999999999999218, 12.50000000000000000, -0.3464101615137741286 ) ) ;
#106905=CARTESIAN_POINT ( 'NONE',  ( 3.349999999999943689, 2.500000000000000000, 2.165063509461097713 ) ) ;
#106906=CARTESIAN_POINT ( 'NONE',  ( -7.100000000000013856, 2.500000000000000000, 5.022947341949748790 ) ) ;
#106907=LINE ( 'NONE', #97739, #114073 ) ;
#106908=DIRECTION ( 'NONE',  ( 0.000000000000000000, 0.000000000000000000, -1.000000000000000000 ) ) ;
#106909=CARTESIAN_POINT ( 'NONE',  ( -1.900000000000034550, 2.500000000000000000, 4.576537180435972019 ) ) ;
#106910=LINE ( 'NONE', #76182, #44991 ) ;
#106911=DIRECTION ( 'NONE',  ( 0.000000000000000000, 0.000000000000000000, 1.000000000000000000 ) ) ;
#106912=CARTESIAN_POINT ( 'NONE',  ( 9.199999999999915801, 2.500000000000000000, -4.330127018922201643 ) ) ;
#106913=EDGE_LOOP ( 'NONE', ( #17649, #14823, #103484, #18543 ) ) ;
#106914=ORIENTED_EDGE ( 'NONE', *, *, #87417, .T. ) ;
#106915=EDGE_LOOP ( 'NONE', ( #79111, #128626 ) ) ;
#106916=ORIENTED_EDGE ( 'NONE', *, *, #81783, .T. ) ;
#106917=DIRECTION ( 'NONE',  ( 0.000000000000000000, 0.000000000000000000, 1.000000000000000000 ) ) ;
#106918=CARTESIAN_POINT ( 'NONE',  ( 2.099999999999947686, 12.50000000000000000, 5.022947341949748790 ) ) ;
#106919=ORIENTED_EDGE ( 'NONE', *, *, #97394, .T. ) ;
#106920=ORIENTED_EDGE ( 'NONE', *, *, #62297, .F. ) ;
#106921=ORIENTED_EDGE ( 'NONE', *, *, #22673, .T. ) ;
#106922=CARTESIAN_POINT ( 'NONE',  ( -3.749999999999991562, 2.500000000000000000, 6.595190528383296780 ) ) ;
#106923=AXIS2_PLACEMENT_3D ( 'NONE', #18123, #86867, #96047 ) ;
#106924=AXIS2_PLACEMENT_3D ( 'NONE', #78822, #29075, #68975 ) ;
#106925=DIRECTION ( 'NONE',  ( 0.000000000000000000, 0.000000000000000000, 1.000000000000000000 ) ) ;
#106926=DIRECTION ( 'NONE',  ( -0.000000000000000000, 1.000000000000000000, -0.000000000000000000 ) ) ;
#106927=FACE_OUTER_BOUND ( 'NONE', #43218, .T. ) ;
#106928=DIRECTION ( 'NONE',  ( 0.000000000000000000, 0.000000000000000000, -1.000000000000000000 ) ) ;
#106929=ORIENTED_EDGE ( 'NONE', *, *, #44545, .F. ) ;
#106930=CIRCLE ( 'NONE', #37987, 0.1000000000000000472 ) ;
#106931=CIRCLE ( 'NONE', #29581, 0.06509327318403745899 ) ;
#106932=ORIENTED_EDGE ( 'NONE', *, *, #120504, .F. ) ;
#106933=EDGE_CURVE ( 'NONE', #50878, #15438, #92472, .T. ) ;
#106934=ORIENTED_EDGE ( 'NONE', *, *, #111544, .T. ) ;
#106936=ORIENTED_EDGE ( 'NONE', *, *, #37558, .F. ) ;
#106937=EDGE_CURVE ( 'NONE', #110796, #59346, #38103, .T. ) ;
#106938=LINE ( 'NONE', #17250, #111089 ) ;
#106939=EDGE_LOOP ( 'NONE', ( #68425, #93868, #75333, #123329 ) ) ;
#106940=EDGE_LOOP ( 'NONE', ( #106644, #88014 ) ) ;
#106941=AXIS2_PLACEMENT_3D ( 'NONE', #84801, #124729, #35082 ) ;
#106942=CARTESIAN_POINT ( 'NONE',  ( -11.25000000000000000, 12.50000000000000000, 2.792790559304612064 ) ) ;
#106943=EDGE_CURVE ( 'NONE', #82416, #102898, #79857, .T. ) ;
#106944=AXIS2_PLACEMENT_3D ( 'NONE', #17182, #116696, #66940 ) ;
#106945=DIRECTION ( 'NONE',  ( 0.000000000000000000, 1.000000000000000000, 0.000000000000000000 ) ) ;
#106946=DIRECTION ( 'NONE',  ( 0.000000000000000000, -0.9999939076577903929, 0.003490651415223739937 ) ) ;
#106947=DIRECTION ( 'NONE',  ( 0.000000000000000000, 0.000000000000000000, 1.000000000000000000 ) ) ;
#106948=CIRCLE ( 'NONE', #19103, 0.1000000000000002554 ) ;
#106949=DIRECTION ( 'NONE',  ( 0.000000000000000000, 0.000000000000000000, 1.000000000000000000 ) ) ;
#106950=AXIS2_PLACEMENT_3D ( 'NONE', #110263, #120095, #112202 ) ;
#106951=ORIENTED_EDGE ( 'NONE', *, *, #52107, .F. ) ;
#106952=DIRECTION ( 'NONE',  ( -0.000000000000000000, 1.000000000000000000, -0.000000000000000000 ) ) ;
#106953=VERTEX_POINT ( 'NONE', #90449 ) ;
#106954=CARTESIAN_POINT ( 'NONE',  ( 0.5999999999999555689, 2.500000000000000000, 4.676537180435972552 ) ) ;
#106955=ORIENTED_EDGE ( 'NONE', *, *, #109535, .F. ) ;
#106956=CARTESIAN_POINT ( 'NONE',  ( 4.149999999999938183, 12.50000000000000000, 5.802370205355744659 ) ) ;
#106957=AXIS2_PLACEMENT_3D ( 'NONE', #118648, #39481, #8675 ) ;
#106958=AXIS2_PLACEMENT_3D ( 'NONE', #20688, #119515, #29859 ) ;
#106959=FACE_OUTER_BOUND ( 'NONE', #113766, .T. ) ;
#106960=ORIENTED_EDGE ( 'NONE', *, *, #87841, .T. ) ;
#106961=CARTESIAN_POINT ( 'NONE',  ( 13.09999999999990195, 2.500000000000000000, 4.776537180435972196 ) ) ;
#106963=ORIENTED_EDGE ( 'NONE', *, *, #120614, .F. ) ;
#106964=DIRECTION ( 'NONE',  ( -4.274815082592931898E-19, -0.9999939076577903929, -0.003490651415223739937 ) ) ;
#106965=ORIENTED_EDGE ( 'NONE', *, *, #5565, .T. ) ;
#106966=ORIENTED_EDGE ( 'NONE', *, *, #13977, .T. ) ;
#106967=DIRECTION ( 'NONE',  ( -0.000000000000000000, -1.000000000000000000, -0.000000000000000000 ) ) ;
#106968=DIRECTION ( 'NONE',  ( 0.000000000000000000, 0.000000000000000000, 1.000000000000000000 ) ) ;
#106970=CARTESIAN_POINT ( 'NONE',  ( -4.150000000000025224, 12.50000000000000000, 6.430097255199259010 ) ) ;
#106971=EDGE_CURVE ( 'NONE', #43111, #12708, #61667, .T. ) ;
#106972=DIRECTION ( 'NONE',  ( -0.000000000000000000, -1.000000000000000000, -0.000000000000000000 ) ) ;
#106973=LINE ( 'NONE', #17290, #61219 ) ;
#106974=VECTOR ( 'NONE', #27484, 1000.000000000000000 ) ;
#106975=AXIS2_PLACEMENT_3D ( 'NONE', #48893, #88798, #50817 ) ;
#106976=AXIS2_PLACEMENT_3D ( 'NONE', #102937, #25031, #65592 ) ;
#106977=ORIENTED_EDGE ( 'NONE', *, *, #64937, .F. ) ;
#106978=DIRECTION ( 'NONE',  ( 0.000000000000000000, 0.000000000000000000, -1.000000000000000000 ) ) ;
#106979=CONICAL_SURFACE ( 'NONE', #86049, 0.1000000000000002554, 0.003490658503988666988 ) ;
#106980=CIRCLE ( 'NONE', #29633, 0.06509327318403745899 ) ;
#106981=EDGE_LOOP ( 'NONE', ( #83191, #91049 ) ) ;
#106982=CIRCLE ( 'NONE', #12889, 0.1000000000000002554 ) ;
#106983=EDGE_CURVE ( 'NONE', #69489, #87658, #65271, .T. ) ;
#106984=CONICAL_SURFACE ( 'NONE', #113260, 0.1000000000000002554, 0.003490658503988666988 ) ;
#106985=DIRECTION ( 'NONE',  ( 0.000000000000000000, 1.000000000000000000, 0.000000000000000000 ) ) ;
#106986=LINE ( 'NONE', #127935, #94937 ) ;
#106987=LINE ( 'NONE', #8148, #50681 ) ;
#106988=EDGE_CURVE ( 'NONE', #13612, #55568, #22393, .T. ) ;
#106989=DIRECTION ( 'NONE',  ( -0.000000000000000000, 1.000000000000000000, -0.000000000000000000 ) ) ;
#106990=CARTESIAN_POINT ( 'NONE',  ( -5.000000000000026645, 2.500000000000000000, -3.637306695894650055 ) ) ;
#106991=EDGE_LOOP ( 'NONE', ( #39085, #60934, #103883, #44145 ) ) ;
#106992=AXIS2_PLACEMENT_3D ( 'NONE', #4980, #44932, #88038 ) ;
#106993=CARTESIAN_POINT ( 'NONE',  ( 12.09999999999990550, 12.50000000000000000, 5.022947341949748790 ) ) ;
#106994=DIRECTION ( 'NONE',  ( 0.000000000000000000, 1.000000000000000000, 0.000000000000000000 ) ) ;
#106995=ADVANCED_FACE ( 'NONE', ( #93692 ), #96564, .T. ) ;
#106996=ORIENTED_EDGE ( 'NONE', *, *, #113838, .F. ) ;
#106997=CARTESIAN_POINT ( 'NONE',  ( -8.350000000000008527, 12.50000000000000000, 5.737276932171707422 ) ) ;
#106998=VERTEX_POINT ( 'NONE', #44594 ) ;
#106999=VERTEX_POINT ( 'NONE', #4008 ) ;
#107000=DIRECTION ( 'NONE',  ( 0.000000000000000000, 0.000000000000000000, 1.000000000000000000 ) ) ;
#107001=ORIENTED_EDGE ( 'NONE', *, *, #90672, .F. ) ;
#107002=CARTESIAN_POINT ( 'NONE',  ( 5.599999999999933031, 2.500000000000000000, -0.4464101615137783252 ) ) ;
#107003=DIRECTION ( 'NONE',  ( -0.000000000000000000, -1.000000000000000000, -0.000000000000000000 ) ) ;
#107004=DIRECTION ( 'NONE',  ( 0.000000000000000000, 1.000000000000000000, 0.000000000000000000 ) ) ;
#107005=AXIS2_PLACEMENT_3D ( 'NONE', #40370, #121475, #119542 ) ;
#107006=ORIENTED_EDGE ( 'NONE', *, *, #60626, .F. ) ;
#107007=CIRCLE ( 'NONE', #33864, 0.06509327318403745899 ) ;
#107008=FACE_BOUND ( 'NONE', #85943, .T. ) ;
#107009=CARTESIAN_POINT ( 'NONE',  ( 4.349999999999940137, 2.500000000000000000, -6.841600689897078702 ) ) ;
#107010=VERTEX_POINT ( 'NONE', #84516 ) ;
#107011=CARTESIAN_POINT ( 'NONE',  ( 8.749999999999921840, 2.500000000000000000, -5.802370205355749988 ) ) ;
#107012=DIRECTION ( 'NONE',  ( 0.000000000000000000, 0.000000000000000000, 1.000000000000000000 ) ) ;
#107013=AXIS2_PLACEMENT_3D ( 'NONE', #33946, #100731, #11057 ) ;
#107014=ORIENTED_EDGE ( 'NONE', *, *, #121051, .F. ) ;
#107015=AXIS2_PLACEMENT_3D ( 'NONE', #75551, #114204, #35023 ) ;
#107016=EDGE_CURVE ( 'NONE', #121453, #65156, #82007, .T. ) ;
#107017=AXIS2_PLACEMENT_3D ( 'NONE', #68355, #75589, #17966 ) ;
#107018=ORIENTED_EDGE ( 'NONE', *, *, #4546, .T. ) ;
#107019=VERTEX_POINT ( 'NONE', #12539 ) ;
#107020=DIRECTION ( 'NONE',  ( 0.000000000000000000, 0.000000000000000000, -1.000000000000000000 ) ) ;
#107021=DIRECTION ( 'NONE',  ( 0.000000000000000000, 0.000000000000000000, 1.000000000000000000 ) ) ;
#107022=FACE_OUTER_BOUND ( 'NONE', #10587, .T. ) ;
#107023=EDGE_CURVE ( 'NONE', #3943, #70330, #2721, .T. ) ;
#107024=FACE_BOUND ( 'NONE', #121807, .T. ) ;
#107025=ORIENTED_EDGE ( 'NONE', *, *, #109734, .T. ) ;
#107026=ADVANCED_FACE ( 'NONE', ( #23023 ), #83239, .T. ) ;
#107027=DIRECTION ( 'NONE',  ( 0.000000000000000000, 0.000000000000000000, 1.000000000000000000 ) ) ;
#107028=DIRECTION ( 'NONE',  ( 0.000000000000000000, 1.000000000000000000, 0.000000000000000000 ) ) ;
#107029=AXIS2_PLACEMENT_3D ( 'NONE', #94298, #116521, #46489 ) ;
#107030=ORIENTED_EDGE ( 'NONE', *, *, #80811, .T. ) ;
#107031=AXIS2_PLACEMENT_3D ( 'NONE', #34790, #125084, #63593 ) ;
#107032=CARTESIAN_POINT ( 'NONE',  ( -11.64999999999999858, 12.50000000000000000, -5.867463478539783672 ) ) ;
#107033=AXIS2_PLACEMENT_3D ( 'NONE', #108808, #129140, #39471 ) ;
#107034=AXIS2_PLACEMENT_3D ( 'NONE', #74129, #53834, #95701 ) ;
#107035=AXIS2_PLACEMENT_3D ( 'NONE', #73433, #31595, #53176 ) ;
#107036=EDGE_CURVE ( 'NONE', #46960, #37231, #46491, .T. ) ;
#107037=CARTESIAN_POINT ( 'NONE',  ( -12.89999999999999147, 2.500000000000000000, -0.6928203230275500335 ) ) ;
#107038=EDGE_CURVE ( 'NONE', #94894, #69453, #98717, .T. ) ;
#107040=ADVANCED_FACE ( 'NONE', ( #42687 ), #55058, .T. ) ;
#107041=PLANE ( 'NONE',  #114036 ) ;
#107042=AXIS2_PLACEMENT_3D ( 'NONE', #93215, #28173, #34301 ) ;
#107043=CARTESIAN_POINT ( 'NONE',  ( -3.350000000000028955, 2.500000000000000000, -2.165063509461101710 ) ) ;
#107044=ADVANCED_FACE ( 'NONE', ( #122512 ), #73587, .T. ) ;
#107045=ORIENTED_EDGE ( 'NONE', *, *, #55522, .T. ) ;
#107046=CONICAL_SURFACE ( 'NONE', #38011, 0.09999999999999982514, 0.003490658503988666988 ) ;
#107047=VERTEX_POINT ( 'NONE', #5295 ) ;
#107048=ORIENTED_EDGE ( 'NONE', *, *, #12470, .T. ) ;
#107049=EDGE_LOOP ( 'NONE', ( #110260, #69840 ) ) ;
#107050=EDGE_LOOP ( 'NONE', ( #84513, #108932 ) ) ;
#107051=FACE_OUTER_BOUND ( 'NONE', #525, .T. ) ;
#107052=DIRECTION ( 'NONE',  ( 0.000000000000000000, 1.000000000000000000, 0.000000000000000000 ) ) ;
#107053=VERTEX_POINT ( 'NONE', #124443 ) ;
#107054=FACE_BOUND ( 'NONE', #30517, .T. ) ;
#107055=EDGE_CURVE ( 'NONE', #53009, #31935, #417, .T. ) ;
#107056=DIRECTION ( 'NONE',  ( 0.000000000000000000, 0.000000000000000000, 1.000000000000000000 ) ) ;
#107057=CARTESIAN_POINT ( 'NONE',  ( 1.049999999999954525, 2.500000000000000000, -2.411473670974877859 ) ) ;
#107058=DIRECTION ( 'NONE',  ( 0.000000000000000000, 1.000000000000000000, 0.000000000000000000 ) ) ;
#107059=CARTESIAN_POINT ( 'NONE',  ( -6.650000000000014566, 12.50000000000000000, 2.099970236277060032 ) ) ;
#107060=DIRECTION ( 'NONE',  ( -4.274815082592931898E-19, -0.9999939076577903929, -0.003490651415223739937 ) ) ;
#107061=VERTEX_POINT ( 'NONE', #74698 ) ;
#107062=DIRECTION ( 'NONE',  ( 0.000000000000000000, 1.000000000000000000, 0.000000000000000000 ) ) ;
#107063=ORIENTED_EDGE ( 'NONE', *, *, #60921, .T. ) ;
#107064=ORIENTED_EDGE ( 'NONE', *, *, #67993, .T. ) ;
#107065=CIRCLE ( 'NONE', #127922, 0.1000000000000002554 ) ;
#107066=EDGE_LOOP ( 'NONE', ( #66856, #49917 ) ) ;
#107067=VECTOR ( 'NONE', #105580, 1000.000000000000000 ) ;
#107068=DIRECTION ( 'NONE',  ( 0.000000000000000000, 1.000000000000000000, 0.000000000000000000 ) ) ;
#107069=CONICAL_SURFACE ( 'NONE', #81937, 0.1000000000000002554, 0.003490658503988666988 ) ;
#107070=DIRECTION ( 'NONE',  ( -0.000000000000000000, -1.000000000000000000, -0.000000000000000000 ) ) ;
#107071=CARTESIAN_POINT ( 'NONE',  ( 0.5999999999999560130, 2.500000000000000000, -3.983716857408426293 ) ) ;
#107072=ORIENTED_EDGE ( 'NONE', *, *, #77491, .F. ) ;
#107073=CARTESIAN_POINT ( 'NONE',  ( 10.87377556642454657, 1.500000000000127676, -8.986829606636716150 ) ) ;
#107074=CARTESIAN_POINT ( 'NONE',  ( -7.900000000000014566, 2.500000000000000000, 0.7928203230275495672 ) ) ;
#107075=CONICAL_SURFACE ( 'NONE', #86135, 0.09999999999999982514, 0.003490658503988666988 ) ;
#107076=CIRCLE ( 'NONE', #121660, 0.06509327318403745899 ) ;
#107077=CARTESIAN_POINT ( 'NONE',  ( 10.84999999999991260, 2.500000000000000000, 5.702370205355745014 ) ) ;
#107079=DIRECTION ( 'NONE',  ( 0.000000000000000000, 0.000000000000000000, 1.000000000000000000 ) ) ;
#107080=DIRECTION ( 'NONE',  ( -0.000000000000000000, 1.000000000000000000, -0.000000000000000000 ) ) ;
#107081=CIRCLE ( 'NONE', #8786, 0.09999999999999982514 ) ;
#107082=CIRCLE ( 'NONE', #109229, 0.1000000000000002554 ) ;
#107083=DIRECTION ( 'NONE',  ( 0.000000000000000000, 0.000000000000000000, 1.000000000000000000 ) ) ;
#107084=EDGE_LOOP ( 'NONE', ( #93251, #57845, #84783, #32701 ) ) ;
#107085=DIRECTION ( 'NONE',  ( 0.000000000000000000, 0.000000000000000000, -1.000000000000000000 ) ) ;
#107086=CIRCLE ( 'NONE', #104928, 0.06509327318403745899 ) ;
#107087=EDGE_LOOP ( 'NONE', ( #19059, #33662, #61744, #16657 ) ) ;
#107088=EDGE_CURVE ( 'NONE', #74853, #63445, #31839, .T. ) ;
#107089=EDGE_LOOP ( 'NONE', ( #103725, #18379, #51209, #15134 ) ) ;
#107091=CARTESIAN_POINT ( 'NONE',  ( 4.149999999999939959, 2.500000000000000000, -6.395190528383301931 ) ) ;
#107092=DIRECTION ( 'NONE',  ( -0.000000000000000000, -1.000000000000000000, -0.000000000000000000 ) ) ;
#107093=ORIENTED_EDGE ( 'NONE', *, *, #47124, .T. ) ;
#107094=ORIENTED_EDGE ( 'NONE', *, *, #116966, .T. ) ;
#107095=AXIS2_PLACEMENT_3D ( 'NONE', #82887, #25223, #65139 ) ;
#107096=ADVANCED_FACE ( 'NONE', ( #24950 ), #25552, .T. ) ;
#107097=CARTESIAN_POINT ( 'NONE',  ( 21.23528140090950700, -2.699413673072311948, -2.293764360948876480 ) ) ;
#107098=CARTESIAN_POINT ( 'NONE',  ( 15.39999999999989200, 2.500000000000000000, 0.6928203230275494784 ) ) ;
#107099=DIRECTION ( 'NONE',  ( 0.000000000000000000, 0.000000000000000000, -1.000000000000000000 ) ) ;
#107100=EDGE_LOOP ( 'NONE', ( #98882, #68873 ) ) ;
#107102=DIRECTION ( 'NONE',  ( 0.000000000000000000, -0.9999939076577903929, 0.003490651415223739937 ) ) ;
#107103=AXIS2_PLACEMENT_3D ( 'NONE', #117434, #127936, #16026 ) ;
#107104=VERTEX_POINT ( 'NONE', #64229 ) ;
#107105=CARTESIAN_POINT ( 'NONE',  ( 1.649999999999948841, 2.500000000000000000, 6.495190528383297135 ) ) ;
#107106=CIRCLE ( 'NONE', #73658, 0.09999999999999982514 ) ;
#107107=FACE_OUTER_BOUND ( 'NONE', #77528, .T. ) ;
#107108=VERTEX_POINT ( 'NONE', #104776 ) ;
#107109=FACE_OUTER_BOUND ( 'NONE', #54341, .T. ) ;
#107110=DIRECTION ( 'NONE',  ( 0.000000000000000000, 0.000000000000000000, -1.000000000000000000 ) ) ;
#107111=CARTESIAN_POINT ( 'NONE',  ( -10.60000000000000320, 12.50000000000000000, -4.611443907251935315 ) ) ;
#107112=DIRECTION ( 'NONE',  ( 0.000000000000000000, 0.000000000000000000, -1.000000000000000000 ) ) ;
#107113=AXIS2_PLACEMENT_3D ( 'NONE', #80957, #52773, #120870 ) ;
#107114=ORIENTED_EDGE ( 'NONE', *, *, #100743, .F. ) ;
#107115=AXIS2_PLACEMENT_3D ( 'NONE', #100960, #832, #10625 ) ;
#107116=DIRECTION ( 'NONE',  ( -0.000000000000000000, -1.000000000000000000, -0.000000000000000000 ) ) ;
#107117=AXIS2_PLACEMENT_3D ( 'NONE', #127294, #118099, #116161 ) ;
#107118=CARTESIAN_POINT ( 'NONE',  ( 1.649999999999951505, 2.500000000000000000, 2.757883832488649656 ) ) ;
#107119=ORIENTED_EDGE ( 'NONE', *, *, #126582, .T. ) ;
#107121=ORIENTED_EDGE ( 'NONE', *, *, #123015, .F. ) ;
#107124=CARTESIAN_POINT ( 'NONE',  ( 0.3999999999999563904, 2.500000000000000000, 5.022947341949748790 ) ) ;
#107125=FACE_OUTER_BOUND ( 'NONE', #104200, .T. ) ;
#107126=AXIS2_PLACEMENT_3D ( 'NONE', #109946, #20909, #11070 ) ;
#107127=LINE ( 'NONE', #36494, #76142 ) ;
#107128=FACE_OUTER_BOUND ( 'NONE', #7667, .T. ) ;
#107129=CONICAL_SURFACE ( 'NONE', #13123, 0.1000000000000002554, 0.003490658503988666988 ) ;
#107130=EDGE_CURVE ( 'NONE', #17899, #84933, #21365, .T. ) ;
#107131=DIRECTION ( 'NONE',  ( 0.000000000000000000, 1.000000000000000000, 0.000000000000000000 ) ) ;
#107132=CIRCLE ( 'NONE', #50707, 0.06509327318403745899 ) ;
#107133=CARTESIAN_POINT ( 'NONE',  ( -2.500000000000032419, 2.500000000000000000, -3.637306695894650055 ) ) ;
#107134=VECTOR ( 'NONE', #32129, 1000.000000000000000 ) ;
#107135=CIRCLE ( 'NONE', #63322, 0.06509327318403745899 ) ;
#107136=CARTESIAN_POINT ( 'NONE',  ( 6.849999999999929479, 12.50000000000000000, -1.818653347947326138 ) ) ;
#107137=AXIS2_PLACEMENT_3D ( 'NONE', #35277, #54887, #64710 ) ;
#107138=CARTESIAN_POINT ( 'NONE',  ( -6.850000000000017408, 12.50000000000000000, -1.818653347947325916 ) ) ;
#107139=EDGE_CURVE ( 'NONE', #10760, #83674, #64862, .T. ) ;
#107140=AXIS2_PLACEMENT_3D ( 'NONE', #110609, #42542, #62175 ) ;
#107141=VERTEX_POINT ( 'NONE', #62313 ) ;
#107142=DIRECTION ( 'NONE',  ( 0.000000000000000000, 0.000000000000000000, 1.000000000000000000 ) ) ;
#107143=EDGE_CURVE ( 'NONE', #55337, #66379, #113402, .T. ) ;
#107144=CARTESIAN_POINT ( 'NONE',  ( 1.449999999999951772, 12.50000000000000000, -6.148780366869526226 ) ) ;
#107145=ADVANCED_FACE ( 'NONE', ( #56969 ), #119750, .T. ) ;
#107146=CARTESIAN_POINT ( 'NONE',  ( 14.19999999999989626, 2.500000000000000000, 0.09999999999999772959 ) ) ;
#107147=CARTESIAN_POINT ( 'NONE',  ( -10.60000000000000320, 2.500000000000000000, -3.983716857408421852 ) ) ;
#107148=EDGE_LOOP ( 'NONE', ( #10782, #81691, #87825, #30075 ) ) ;
#107149=CARTESIAN_POINT ( 'NONE',  ( -10.20000000000000462, 12.50000000000000000, -4.676537180435973440 ) ) ;
#107150=EDGE_CURVE ( 'NONE', #98294, #106877, #77904, .T. ) ;
#107152=DIRECTION ( 'NONE',  ( 0.000000000000000000, 0.000000000000000000, 1.000000000000000000 ) ) ;
#107153=ORIENTED_EDGE ( 'NONE', *, *, #103650, .F. ) ;
#107154=CIRCLE ( 'NONE', #19324, 0.1000000000000000056 ) ;
#107155=EDGE_CURVE ( 'NONE', #118854, #93025, #42403, .T. ) ;
#107156=ORIENTED_EDGE ( 'NONE', *, *, #28, .F. ) ;
#107157=VERTEX_POINT ( 'NONE', #96250 ) ;
#107158=EDGE_LOOP ( 'NONE', ( #81229, #55994, #111199, #41842 ) ) ;
#107159=AXIS2_PLACEMENT_3D ( 'NONE', #57963, #27843, #97870 ) ;
#107160=ORIENTED_EDGE ( 'NONE', *, *, #60831, .T. ) ;
#107161=DIRECTION ( 'NONE',  ( -0.000000000000000000, -1.000000000000000000, -0.000000000000000000 ) ) ;
#107162=CIRCLE ( 'NONE', #11017, 0.09999999999999999167 ) ;
#107163=CIRCLE ( 'NONE', #67427, 0.1000000000000002554 ) ;
#107164=DIRECTION ( 'NONE',  ( 0.000000000000000000, 1.000000000000000000, 0.000000000000000000 ) ) ;
#107165=CARTESIAN_POINT ( 'NONE',  ( -10.00000000000000533, 2.500000000000000000, -4.922947341949749145 ) ) ;
#107166=DIRECTION ( 'NONE',  ( 0.000000000000000000, 0.000000000000000000, 1.000000000000000000 ) ) ;
#107167=CONICAL_SURFACE ( 'NONE', #82040, 0.1000000000000002554, 0.003490658503988666988 ) ;
#107168=ORIENTED_EDGE ( 'NONE', *, *, #97858, .F. ) ;
#107169=CIRCLE ( 'NONE', #34027, 0.09999999999999982514 ) ;
#107170=AXIS2_PLACEMENT_3D ( 'NONE', #93957, #23262, #82862 ) ;
#107171=CARTESIAN_POINT ( 'NONE',  ( 7.299999999999926104, 12.50000000000000000, -3.983716857408426293 ) ) ;
#107172=AXIS2_PLACEMENT_3D ( 'NONE', #126909, #67299, #62988 ) ;
#107173=ORIENTED_EDGE ( 'NONE', *, *, #77024, .F. ) ;
#107174=CARTESIAN_POINT ( 'NONE',  ( 76.45227062060567391, -3.905198618290971257, -5.870121734780581413 ) ) ;
#107175=FACE_OUTER_BOUND ( 'NONE', #99109, .T. ) ;
#107176=CONICAL_SURFACE ( 'NONE', #88383, 0.09999999999999982514, 0.003490658503988666988 ) ;
#107177=DIRECTION ( 'NONE',  ( -0.000000000000000000, -1.000000000000000000, -0.000000000000000000 ) ) ;
#107178=CIRCLE ( 'NONE', #11027, 0.09999999999999982514 ) ;
#107179=FACE_OUTER_BOUND ( 'NONE', #73489, .T. ) ;
#107180=CARTESIAN_POINT ( 'NONE',  ( -11.04999999999999893, 12.50000000000000000, 6.148780366869520009 ) ) ;
#107181=CONICAL_SURFACE ( 'NONE', #50766, 0.09999999999999982514, 0.003490658503988666988 ) ;
#107182=ORIENTED_EDGE ( 'NONE', *, *, #82734, .F. ) ;
#107183=ADVANCED_FACE ( 'NONE', ( #106718 ), #103019, .T. ) ;
#107185=ORIENTED_EDGE ( 'NONE', *, *, #16553, .T. ) ;
#107187=CARTESIAN_POINT ( 'NONE',  ( -3.642919299551294898E-14, 12.50000000000000000, 0.6928203230275518099 ) ) ;
#107188=DIRECTION ( 'NONE',  ( 0.000000000000000000, 0.000000000000000000, 1.000000000000000000 ) ) ;
#107189=CARTESIAN_POINT ( 'NONE',  ( -12.09999999999999609, 2.500000000000000000, -4.330127018922198978 ) ) ;
#107190=ADVANCED_FACE ( 'NONE', ( #97551 ), #23608, .T. ) ;
#107191=FACE_BOUND ( 'NONE', #123021, .T. ) ;
#107192=CARTESIAN_POINT ( 'NONE',  ( -14.34999999999998543, 2.500000000000000000, 2.411473670974877415 ) ) ;
#107193=CARTESIAN_POINT ( 'NONE',  ( -12.04999999999999538, 12.50000000000000000, 2.099970236277060032 ) ) ;
#107194=ADVANCED_FACE ( 'NONE', ( #15759 ), #27711, .T. ) ;
#107195=DIRECTION ( 'NONE',  ( -0.000000000000000000, 1.000000000000000000, -0.000000000000000000 ) ) ;
#107196=CARTESIAN_POINT ( 'NONE',  ( -2.700000000000030820, 12.50000000000000000, 0.3464101615137735735 ) ) ;
#107197=CIRCLE ( 'NONE', #84205, 0.06509327318403743123 ) ;
#107198=EDGE_CURVE ( 'NONE', #92191, #60850, #31937, .T. ) ;
#107202=DIRECTION ( 'NONE',  ( 0.000000000000000000, -0.9999939076577903929, 0.003490651415223739937 ) ) ;
#107203=ADVANCED_FACE ( 'NONE', ( #86438 ), #36064, .T. ) ;
#107204=AXIS2_PLACEMENT_3D ( 'NONE', #74817, #55178, #6055 ) ;
#107205=AXIS2_PLACEMENT_3D ( 'NONE', #29159, #67770, #18672 ) ;
#107206=CIRCLE ( 'NONE', #123926, 0.1000000000000000472 ) ;
#107207=CARTESIAN_POINT ( 'NONE',  ( -10.40000000000000213, 2.500000000000000000, -4.430127018922197735 ) ) ;
#107208=EDGE_CURVE ( 'NONE', #35207, #78590, #117822, .T. ) ;
#107209=ORIENTED_EDGE ( 'NONE', *, *, #69574, .T. ) ;
#107210=VERTEX_POINT ( 'NONE', #105452 ) ;
#107211=ORIENTED_EDGE ( 'NONE', *, *, #487, .T. ) ;
#107212=ORIENTED_EDGE ( 'NONE', *, *, #108359, .T. ) ;
#107213=CARTESIAN_POINT ( 'NONE',  ( 13.09999999999990195, 12.50000000000000000, 4.676537180435972552 ) ) ;
#107214=FACE_BOUND ( 'NONE', #85486, .T. ) ;
#107215=VECTOR ( 'NONE', #77888, 1000.000000000000000 ) ;
#107216=DIRECTION ( 'NONE',  ( 0.000000000000000000, 1.000000000000000000, 0.000000000000000000 ) ) ;
#107217=CIRCLE ( 'NONE', #128159, 0.09999999999999982514 ) ;
#107218=EDGE_CURVE ( 'NONE', #117937, #10213, #88335, .T. ) ;
#107219=LINE ( 'NONE', #86930, #41454 ) ;
#107220=CIRCLE ( 'NONE', #75916, 0.06509327318403745899 ) ;
#107221=ADVANCED_FACE ( 'NONE', ( #27503 ), #67417, .T. ) ;
#107222=ORIENTED_EDGE ( 'NONE', *, *, #3600, .T. ) ;
#107223=DIRECTION ( 'NONE',  ( 0.000000000000000000, 1.000000000000000000, 0.000000000000000000 ) ) ;
#107224=CARTESIAN_POINT ( 'NONE',  ( -5.000000000000024869, 2.500000000000000000, -5.122947341949753763 ) ) ;
#107225=FACE_OUTER_BOUND ( 'NONE', #75304, .T. ) ;
#107226=VERTEX_POINT ( 'NONE', #36720 ) ;
#107228=DIRECTION ( 'NONE',  ( 0.000000000000000000, 1.000000000000000000, 0.000000000000000000 ) ) ;
#107229=CIRCLE ( 'NONE', #48560, 0.1000000000000002554 ) ;
#107230=CIRCLE ( 'NONE', #94710, 0.06509327318403745899 ) ;
#107231=AXIS2_PLACEMENT_3D ( 'NONE', #98107, #18262, #7136 ) ;
#107232=CIRCLE ( 'NONE', #65460, 0.06509327318403745899 ) ;
#107233=ORIENTED_EDGE ( 'NONE', *, *, #79081, .T. ) ;
#107234=CARTESIAN_POINT ( 'NONE',  ( -6.050000000000022027, 12.50000000000000000, -1.883746621131363597 ) ) ;
#107235=DIRECTION ( 'NONE',  ( 0.000000000000000000, 0.000000000000000000, -1.000000000000000000 ) ) ;
#107236=VECTOR ( 'NONE', #61349, 1000.000000000000000 ) ;
#107237=ORIENTED_EDGE ( 'NONE', *, *, #56687, .F. ) ;
#107238=DIRECTION ( 'NONE',  ( 0.000000000000000000, -0.000000000000000000, 1.000000000000000000 ) ) ;
#107239=AXIS2_PLACEMENT_3D ( 'NONE', #486, #11610, #51557 ) ;
#107240=CARTESIAN_POINT ( 'NONE',  ( 8.749999999999953815, 12.50000000000000000, 6.430097255199259010 ) ) ;
#107241=CARTESIAN_POINT ( 'NONE',  ( 7.499999999999925393, 2.500000000000000000, -3.637306695894650055 ) ) ;
#107242=EDGE_LOOP ( 'NONE', ( #23086, #85488 ) ) ;
#107243=EDGE_LOOP ( 'NONE', ( #101472, #11045 ) ) ;
#107244=ADVANCED_FACE ( 'NONE', ( #108015 ), #33987, .T. ) ;
#107245=CARTESIAN_POINT ( 'NONE',  ( -3.950000000000026379, 12.50000000000000000, -1.818653347947326138 ) ) ;
#107246=ORIENTED_EDGE ( 'NONE', *, *, #101408, .F. ) ;
#107247=DIRECTION ( 'NONE',  ( -0.000000000000000000, -1.000000000000000000, -0.000000000000000000 ) ) ;
#107248=FACE_BOUND ( 'NONE', #31885, .T. ) ;
#107249=ORIENTED_EDGE ( 'NONE', *, *, #20665, .T. ) ;
#107250=EDGE_CURVE ( 'NONE', #38503, #68589, #28180, .T. ) ;
#107252=VERTEX_POINT ( 'NONE', #95629 ) ;
#107253=DIRECTION ( 'NONE',  ( 0.000000000000000000, -0.9999939076577903929, 0.003490651415223739937 ) ) ;
#107254=FACE_OUTER_BOUND ( 'NONE', #84770, .T. ) ;
#107255=AXIS2_PLACEMENT_3D ( 'NONE', #2621, #22934, #123678 ) ;
#107256=CARTESIAN_POINT ( 'NONE',  ( 7.499999999999927169, 2.500000000000000000, 3.737306695894644371 ) ) ;
#107257=DIRECTION ( 'NONE',  ( -0.000000000000000000, 1.000000000000000000, -0.000000000000000000 ) ) ;
#107259=ORIENTED_EDGE ( 'NONE', *, *, #120914, .F. ) ;
#107260=ADVANCED_FACE ( 'NONE', ( #76635 ), #107129, .T. ) ;
#107261=ORIENTED_EDGE ( 'NONE', *, *, #108968, .T. ) ;
#107262=CARTESIAN_POINT ( 'NONE',  ( 10.39999999999991509, 2.500000000000000000, -0.5928203230275542746 ) ) ;
#107263=AXIS2_PLACEMENT_3D ( 'NONE', #85441, #33762, #84798 ) ;
#107264=CARTESIAN_POINT ( 'NONE',  ( -13.34999999999999076, 2.500000000000000000, -2.757883832488651876 ) ) ;
#107265=CIRCLE ( 'NONE', #128210, 0.06509327318403741736 ) ;
#107266=CARTESIAN_POINT ( 'NONE',  ( -6.050000000000022027, 2.500000000000000000, -1.818653347947326138 ) ) ;
#107267=VERTEX_POINT ( 'NONE', #25576 ) ;
#107268=ORIENTED_EDGE ( 'NONE', *, *, #33484, .T. ) ;
#107269=ORIENTED_EDGE ( 'NONE', *, *, #83289, .T. ) ;
#107270=CARTESIAN_POINT ( 'NONE',  ( -1.450000000000035927, 12.50000000000000000, -6.083687093685488989 ) ) ;
#107271=CARTESIAN_POINT ( 'NONE',  ( -11.24999999999999822, 12.50000000000000000, 5.802370205355744659 ) ) ;
#107272=VECTOR ( 'NONE', #108586, 1000.000000000000000 ) ;
#107273=VECTOR ( 'NONE', #116965, 1000.000000000000000 ) ;
#107274=DIRECTION ( 'NONE',  ( 0.000000000000000000, 0.000000000000000000, 1.000000000000000000 ) ) ;
#107275=AXIS2_PLACEMENT_3D ( 'NONE', #99120, #19916, #9446 ) ;
#107276=DIRECTION ( 'NONE',  ( 0.000000000000000000, 1.000000000000000000, 0.000000000000000000 ) ) ;
#107277=FACE_OUTER_BOUND ( 'NONE', #109668, .T. ) ;
#107278=FACE_OUTER_BOUND ( 'NONE', #4774, .T. ) ;
#107279=DIRECTION ( 'NONE',  ( -0.000000000000000000, 1.000000000000000000, -0.000000000000000000 ) ) ;
#107280=LINE ( 'NONE', #96805, #124070 ) ;
#107281=FACE_OUTER_BOUND ( 'NONE', #54884, .T. ) ;
#107282=AXIS2_PLACEMENT_3D ( 'NONE', #96345, #66248, #65609 ) ;
#107283=ORIENTED_EDGE ( 'NONE', *, *, #63595, .T. ) ;
#107285=CARTESIAN_POINT ( 'NONE',  ( 0.8499999999999527933, 2.500000000000000000, 7.088010851410848190 ) ) ;
#107286=EDGE_LOOP ( 'NONE', ( #67965, #96684 ) ) ;
#107288=DIRECTION ( 'NONE',  ( 0.000000000000000000, -0.000000000000000000, 1.000000000000000000 ) ) ;
#107289=DIRECTION ( 'NONE',  ( -0.000000000000000000, 1.000000000000000000, -0.000000000000000000 ) ) ;
#107290=LINE ( 'NONE', #116459, #109223 ) ;
#107291=AXIS2_PLACEMENT_3D ( 'NONE', #106232, #37503, #76773 ) ;
#107292=DIRECTION ( 'NONE',  ( 0.000000000000000000, 1.000000000000000000, 0.000000000000000000 ) ) ;
#107293=CARTESIAN_POINT ( 'NONE',  ( -11.64999999999999680, 2.500000000000000000, 1.372243186433545370 ) ) ;
#107294=CARTESIAN_POINT ( 'NONE',  ( -12.49999999999999289, 12.50000000000000000, 3.637306695894644726 ) ) ;
#107295=DIRECTION ( 'NONE',  ( -4.274815082592931898E-19, -0.9999939076577903929, -0.003490651415223739937 ) ) ;
#107296=EDGE_LOOP ( 'NONE', ( #88813, #57181 ) ) ;
#107297=CARTESIAN_POINT ( 'NONE',  ( -1.450000000000035927, 12.50000000000000000, -6.148780366869526226 ) ) ;
#107298=CIRCLE ( 'NONE', #67574, 0.06509327318403745899 ) ;
#107299=CARTESIAN_POINT ( 'NONE',  ( -6.505213034913026604E-15, 12.50000000000000000, 4.330127018922196314 ) ) ;
#107300=CIRCLE ( 'NONE', #21631, 0.06509327318403745899 ) ;
#107301=ADVANCED_FACE ( 'NONE', ( #85793 ), #125705, .T. ) ;
#107302=CONICAL_SURFACE ( 'NONE', #11151, 0.1000000000000002554, 0.003490658503988666988 ) ;
#107303=EDGE_LOOP ( 'NONE', ( #18930, #55124, #62331, #127204 ) ) ;
#107304=VERTEX_POINT ( 'NONE', #51056 ) ;
#107305=ADVANCED_FACE ( 'NONE', ( #81153, #41238 ), #50388, .T. ) ;
#107306=VERTEX_POINT ( 'NONE', #78587 ) ;
#107307=EDGE_LOOP ( 'NONE', ( #4033, #25203 ) ) ;
#107308=EDGE_CURVE ( 'NONE', #109714, #127460, #98817, .T. ) ;
#107309=PLANE ( 'NONE',  #8620 ) ;
#107310=DIRECTION ( 'NONE',  ( 0.000000000000000000, -0.9999939076577903929, 0.003490651415223739937 ) ) ;
#107311=CONICAL_SURFACE ( 'NONE', #71818, 0.1000000000000002554, 0.003490658503988666988 ) ;
#107312=AXIS2_PLACEMENT_3D ( 'NONE', #114332, #62195, #5013 ) ;
#107313=ORIENTED_EDGE ( 'NONE', *, *, #86080, .F. ) ;
#107314=CARTESIAN_POINT ( 'NONE',  ( -14.59999999999998366, 2.500000000000000000, -0.7928203230275520097 ) ) ;
#107315=CIRCLE ( 'NONE', #50889, 0.1000000000000000472 ) ;
#107316=CARTESIAN_POINT ( 'NONE',  ( 9.349999999999916156, 2.500000000000000000, -2.411473670974877859 ) ) ;
#107317=ADVANCED_FACE ( 'NONE', ( #11092 ), #50704, .T. ) ;
#107318=DIRECTION ( 'NONE',  ( 0.000000000000000000, 0.000000000000000000, 1.000000000000000000 ) ) ;
#107319=EDGE_CURVE ( 'NONE', #99172, #21324, #1287, .T. ) ;
#107320=ORIENTED_EDGE ( 'NONE', *, *, #49406, .F. ) ;
#107321=ADVANCED_FACE ( 'NONE', ( #118477 ), #40251, .T. ) ;
#107322=CARTESIAN_POINT ( 'NONE',  ( -3.950000000000026379, 12.50000000000000000, 6.841600689897072485 ) ) ;
#107323=VECTOR ( 'NONE', #49147, 1000.000000000000000 ) ;
#107324=FACE_OUTER_BOUND ( 'NONE', #108220, .T. ) ;
#107325=ORIENTED_EDGE ( 'NONE', *, *, #17486, .F. ) ;
#107326=CIRCLE ( 'NONE', #59231, 0.06509327318403745899 ) ;
#107327=VECTOR ( 'NONE', #96619, 1000.000000000000000 ) ;
#107328=ORIENTED_EDGE ( 'NONE', *, *, #30641, .F. ) ;
#107329=ORIENTED_EDGE ( 'NONE', *, *, #122704, .F. ) ;
#107330=FACE_OUTER_BOUND ( 'NONE', #13687, .T. ) ;
#107331=AXIS2_PLACEMENT_3D ( 'NONE', #73568, #91292, #113505 ) ;
#107332=DIRECTION ( 'NONE',  ( 0.000000000000000000, 1.000000000000000000, 0.000000000000000000 ) ) ;
#107333=ORIENTED_EDGE ( 'NONE', *, *, #102393, .T. ) ;
#107334=DIRECTION ( 'NONE',  ( 0.000000000000000000, 0.000000000000000000, 1.000000000000000000 ) ) ;
#107335=DIRECTION ( 'NONE',  ( -0.000000000000000000, 1.000000000000000000, -0.000000000000000000 ) ) ;
#107336=DIRECTION ( 'NONE',  ( 0.000000000000000000, 0.000000000000000000, 1.000000000000000000 ) ) ;
#107337=DIRECTION ( 'NONE',  ( -0.000000000000000000, 1.000000000000000000, -0.000000000000000000 ) ) ;
#107338=ORIENTED_EDGE ( 'NONE', *, *, #119874, .F. ) ;
#107339=DIRECTION ( 'NONE',  ( 0.000000000000000000, 0.000000000000000000, -1.000000000000000000 ) ) ;
#107340=ORIENTED_EDGE ( 'NONE', *, *, #72377, .F. ) ;
#107341=ORIENTED_EDGE ( 'NONE', *, *, #31751, .F. ) ;
#107342=CARTESIAN_POINT ( 'NONE',  ( 0.5999999999999551248, 12.50000000000000000, -4.676537180435978769 ) ) ;
#107343=CIRCLE ( 'NONE', #119872, 0.1000000000000002554 ) ;
#107344=CIRCLE ( 'NONE', #30003, 0.1000000000000000472 ) ;
#107345=CARTESIAN_POINT ( 'NONE',  ( -7.900000000000014566, 2.500000000000000000, -2.276824562219559311E-15 ) ) ;
#107346=FACE_BOUND ( 'NONE', #86659, .T. ) ;
#107348=DIRECTION ( 'NONE',  ( 0.000000000000000000, -0.9999939076577903929, 0.003490651415223739937 ) ) ;
#107350=AXIS2_PLACEMENT_3D ( 'NONE', #83987, #102992, #55198 ) ;
#107351=AXIS2_PLACEMENT_3D ( 'NONE', #66562, #77672, #78348 ) ;
#107352=AXIS2_PLACEMENT_3D ( 'NONE', #37726, #68457, #27901 ) ;
#107353=AXIS2_PLACEMENT_3D ( 'NONE', #40185, #127913, #89914 ) ;
#107354=ADVANCED_FACE ( 'NONE', ( #90295 ), #2659, .T. ) ;
#107355=ORIENTED_EDGE ( 'NONE', *, *, #13929, .T. ) ;
#107356=EDGE_CURVE ( 'NONE', #32515, #89688, #86284, .T. ) ;
#107357=DIRECTION ( 'NONE',  ( 0.000000000000000000, 1.000000000000000000, 0.000000000000000000 ) ) ;
#107358=LINE ( 'NONE', #27485, #82456 ) ;
#107359=CARTESIAN_POINT ( 'NONE',  ( 9.149999999999915090, 2.500000000000000000, -2.065063509461102065 ) ) ;
#107360=ADVANCED_FACE ( 'NONE', ( #49123 ), #67395, .T. ) ;
#107361=FACE_OUTER_BOUND ( 'NONE', #19511, .T. ) ;
#107362=EDGE_LOOP ( 'NONE', ( #111213, #8012, #56768, #83350 ) ) ;
#107363=FACE_OUTER_BOUND ( 'NONE', #105086, .T. ) ;
#107364=VECTOR ( 'NONE', #13233, 1000.000000000000000 ) ;
#107365=AXIS2_PLACEMENT_3D ( 'NONE', #51373, #41553, #91277 ) ;
#107366=CARTESIAN_POINT ( 'NONE',  ( 6.649999999999930189, 2.500000000000000000, -1.472243186433550122 ) ) ;
#107367=EDGE_CURVE ( 'NONE', #65580, #16616, #23509, .T. ) ;
#107368=EDGE_CURVE ( 'NONE', #2989, #54526, #96658, .T. ) ;
#107369=ORIENTED_EDGE ( 'NONE', *, *, #104165, .F. ) ;
#107370=AXIS2_PLACEMENT_3D ( 'NONE', #14391, #105371, #15678 ) ;
#107371=DIRECTION ( 'NONE',  ( 0.000000000000000000, 0.000000000000000000, 1.000000000000000000 ) ) ;
#107372=DIRECTION ( 'NONE',  ( -4.274815082592931898E-19, -0.9999939076577903929, -0.003490651415223739937 ) ) ;
#107373=FACE_BOUND ( 'NONE', #81154, .T. ) ;
#107374=CARTESIAN_POINT ( 'NONE',  ( 8.328334240990686865, -2.500000000000000000, -8.539519492767929876 ) ) ;
#107375=EDGE_CURVE ( 'NONE', #8229, #112688, #69378, .T. ) ;
#107376=EDGE_CURVE ( 'NONE', #125682, #44204, #4710, .T. ) ;
#107377=ORIENTED_EDGE ( 'NONE', *, *, #19684, .F. ) ;
#107378=DIRECTION ( 'NONE',  ( -0.000000000000000000, -1.000000000000000000, -0.000000000000000000 ) ) ;
#107379=EDGE_LOOP ( 'NONE', ( #37846, #114184 ) ) ;
#107380=ORIENTED_EDGE ( 'NONE', *, *, #35577, .T. ) ;
#107381=CARTESIAN_POINT ( 'NONE',  ( 20.37757664703743998, 0.6627606010239225354, -4.188167776336756631 ) ) ;
#107383=ADVANCED_FACE ( 'NONE', ( #30129 ), #21461, .T. ) ;
#107384=AXIS2_PLACEMENT_3D ( 'NONE', #74037, #44579, #51828 ) ;
#107385=ORIENTED_EDGE ( 'NONE', *, *, #50647, .T. ) ;
#107386=DIRECTION ( 'NONE',  ( 0.000000000000000000, -0.9999939076577903929, 0.003490651415223739937 ) ) ;
#107387=DIRECTION ( 'NONE',  ( 0.000000000000000000, 1.000000000000000000, 0.000000000000000000 ) ) ;
#107388=CARTESIAN_POINT ( 'NONE',  ( 4.349999999999936584, 12.50000000000000000, 6.148780366869520009 ) ) ;
#107389=AXIS2_PLACEMENT_3D ( 'NONE', #66602, #27973, #68534 ) ;
#107390=CIRCLE ( 'NONE', #98988, 0.06509327318403745899 ) ;
#107391=CIRCLE ( 'NONE', #117747, 0.1000000000000002554 ) ;
#107392=ORIENTED_EDGE ( 'NONE', *, *, #20915, .T. ) ;
#107393=DIRECTION ( 'NONE',  ( 0.000000000000000000, 0.000000000000000000, 1.000000000000000000 ) ) ;
#107394=CARTESIAN_POINT ( 'NONE',  ( -8.350000000000010303, 12.50000000000000000, 6.495190528383297135 ) ) ;
#107395=CARTESIAN_POINT ( 'NONE',  ( -11.44999999999999929, 2.500000000000000000, -1.818653347947322141 ) ) ;
#107396=DIRECTION ( 'NONE',  ( -0.000000000000000000, 1.000000000000000000, -0.000000000000000000 ) ) ;
#107397=ORIENTED_EDGE ( 'NONE', *, *, #14507, .F. ) ;
#107398=DIRECTION ( 'NONE',  ( 0.000000000000000000, 1.000000000000000000, 0.000000000000000000 ) ) ;
#107399=ORIENTED_EDGE ( 'NONE', *, *, #80923, .F. ) ;
#107400=AXIS2_PLACEMENT_3D ( 'NONE', #79056, #9654, #109120 ) ;
#107401=DIRECTION ( 'NONE',  ( -4.274815082592931898E-19, -0.9999939076577903929, -0.003490651415223739937 ) ) ;
#107402=AXIS2_PLACEMENT_3D ( 'NONE', #24552, #75576, #103765 ) ;
#107403=ORIENTED_EDGE ( 'NONE', *, *, #22655, .T. ) ;
#107404=CONICAL_SURFACE ( 'NONE', #82718, 0.09999999999999982514, 0.003490658503988666988 ) ;
#107405=FACE_OUTER_BOUND ( 'NONE', #27822, .T. ) ;
#107406=LINE ( 'NONE', #25611, #45281 ) ;
#107407=VECTOR ( 'NONE', #121484, 1000.000000000000000 ) ;
#107408=DIRECTION ( 'NONE',  ( -0.000000000000000000, 1.000000000000000000, -0.000000000000000000 ) ) ;
#107409=CARTESIAN_POINT ( 'NONE',  ( 10.59999999999991260, 12.50000000000000000, -0.4115034346978157509 ) ) ;
#107410=ORIENTED_EDGE ( 'NONE', *, *, #91362, .F. ) ;
#107411=DIRECTION ( 'NONE',  ( -0.000000000000000000, -1.000000000000000000, -0.000000000000000000 ) ) ;
#107412=DIRECTION ( 'NONE',  ( 0.000000000000000000, 0.000000000000000000, 1.000000000000000000 ) ) ;
#107413=FACE_OUTER_BOUND ( 'NONE', #127661, .T. ) ;
#107414=DIRECTION ( 'NONE',  ( 0.000000000000000000, 0.000000000000000000, 1.000000000000000000 ) ) ;
#107415=CARTESIAN_POINT ( 'NONE',  ( 14.14999999999989555, 12.50000000000000000, 2.165063509461097713 ) ) ;
#107416=ORIENTED_EDGE ( 'NONE', *, *, #36335, .T. ) ;
#107417=ADVANCED_FACE ( 'NONE', ( #110597 ), #71634, .T. ) ;
#107418=ORIENTED_EDGE ( 'NONE', *, *, #102843, .F. ) ;
#107419=DIRECTION ( 'NONE',  ( 0.000000000000000000, 0.000000000000000000, 1.000000000000000000 ) ) ;
#107420=AXIS2_PLACEMENT_3D ( 'NONE', #76779, #74200, #34934 ) ;
#107421=ORIENTED_EDGE ( 'NONE', *, *, #92829, .F. ) ;
#107422=CONICAL_SURFACE ( 'NONE', #92762, 0.1000000000000002554, 0.003490658503988666988 ) ;
#107423=DIRECTION ( 'NONE',  ( -0.000000000000000000, 1.000000000000000000, -0.000000000000000000 ) ) ;
#107424=VERTEX_POINT ( 'NONE', #86207 ) ;
#107425=ORIENTED_EDGE ( 'NONE', *, *, #47822, .F. ) ;
#107426=ORIENTED_EDGE ( 'NONE', *, *, #94284, .T. ) ;
#107427=CIRCLE ( 'NONE', #103225, 0.09999999999999982514 ) ;
#107428=CARTESIAN_POINT ( 'NONE',  ( -1.250000000000001110, 2.500000000000000000, -6.495190528383302464 ) ) ;
#107429=AXIS2_PLACEMENT_3D ( 'NONE', #34304, #114137, #24467 ) ;
#107430=CARTESIAN_POINT ( 'NONE',  ( 12.29999999999990301, 2.500000000000000000, -0.3464101615137782364 ) ) ;
#107431=CARTESIAN_POINT ( 'NONE',  ( -9.600000000000008527, 2.500000000000000000, -5.122947341949750211 ) ) ;
#107433=FACE_OUTER_BOUND ( 'NONE', #78005, .T. ) ;
#107434=CARTESIAN_POINT ( 'NONE',  ( 4.599999999999940137, 2.500000000000000000, -4.330127018922201643 ) ) ;
#107435=DIRECTION ( 'NONE',  ( 0.000000000000000000, -0.000000000000000000, 1.000000000000000000 ) ) ;
#107436=LINE ( 'NONE', #5508, #101204 ) ;
#107437=EDGE_LOOP ( 'NONE', ( #68304, #109401, #60286, #52404 ) ) ;
#107438=DIRECTION ( 'NONE',  ( 0.000000000000000000, 1.000000000000000000, 0.000000000000000000 ) ) ;
#107439=EDGE_LOOP ( 'NONE', ( #54471, #110282 ) ) ;
#107440=ORIENTED_EDGE ( 'NONE', *, *, #90789, .T. ) ;
#107441=ORIENTED_EDGE ( 'NONE', *, *, #103710, .T. ) ;
#107442=EDGE_LOOP ( 'NONE', ( #93949, #87647, #67190, #85153 ) ) ;
#107443=DIRECTION ( 'NONE',  ( 0.000000000000000000, 0.000000000000000000, 1.000000000000000000 ) ) ;
#107444=AXIS2_PLACEMENT_3D ( 'NONE', #94724, #75723, #16785 ) ;
#107445=AXIS2_PLACEMENT_3D ( 'NONE', #16258, #126241, #84380 ) ;
#107446=ORIENTED_EDGE ( 'NONE', *, *, #20746, .T. ) ;
#107447=EDGE_LOOP ( 'NONE', ( #82685, #18027 ) ) ;
#107448=AXIS2_PLACEMENT_3D ( 'NONE', #86575, #96386, #6692 ) ;
#107449=CARTESIAN_POINT ( 'NONE',  ( -0.8500000000000395017, 2.500000000000000000, 6.495190528383297135 ) ) ;
#107450=CARTESIAN_POINT ( 'NONE',  ( 3.349999999999941913, 12.50000000000000000, 5.802370205355744659 ) ) ;
#107451=CIRCLE ( 'NONE', #42634, 0.06509327318403741736 ) ;
#107452=FACE_OUTER_BOUND ( 'NONE', #93358, .T. ) ;
#107453=CARTESIAN_POINT ( 'NONE',  ( 1.899999999999951283, 12.50000000000000000, -4.676537180435977881 ) ) ;
#107454=AXIS2_PLACEMENT_3D ( 'NONE', #39685, #88756, #79585 ) ;
#107455=DIRECTION ( 'NONE',  ( 0.000000000000000000, 0.000000000000000000, 1.000000000000000000 ) ) ;
#107456=ORIENTED_EDGE ( 'NONE', *, *, #123010, .T. ) ;
#107457=CARTESIAN_POINT ( 'NONE',  ( 2.099999999999948574, 2.500000000000000000, 4.230127018922196669 ) ) ;
#107458=CIRCLE ( 'NONE', #86524, 0.06509327318403745899 ) ;
#107459=AXIS2_PLACEMENT_3D ( 'NONE', #55116, #25637, #7283 ) ;
#107460=ORIENTED_EDGE ( 'NONE', *, *, #42162, .F. ) ;
#107461=FACE_OUTER_BOUND ( 'NONE', #42989, .T. ) ;
#107462=AXIS2_PLACEMENT_3D ( 'NONE', #64236, #44601, #15102 ) ;
#107463=ADVANCED_FACE ( 'NONE', ( #28606 ), #46300, .T. ) ;
#107464=ORIENTED_EDGE ( 'NONE', *, *, #99814, .F. ) ;
#107465=DIRECTION ( 'NONE',  ( 0.000000000000000000, 0.000000000000000000, 1.000000000000000000 ) ) ;
#107466=ORIENTED_EDGE ( 'NONE', *, *, #93320, .T. ) ;
#107467=ADVANCED_FACE ( 'NONE', ( #7651 ), #8728, .T. ) ;
#107468=VERTEX_POINT ( 'NONE', #97333 ) ;
#107469=EDGE_CURVE ( 'NONE', #106056, #123660, #123652, .T. ) ;
#107470=DIRECTION ( 'NONE',  ( 0.000000000000000000, 0.000000000000000000, 1.000000000000000000 ) ) ;
#107471=LINE ( 'NONE', #55156, #75624 ) ;
#107473=PLANE ( 'NONE',  #2597 ) ;
#107474=AXIS2_PLACEMENT_3D ( 'NONE', #87928, #118048, #98400 ) ;
#107475=EDGE_CURVE ( 'NONE', #108499, #59648, #68511, .T. ) ;
#107476=FACE_OUTER_BOUND ( 'NONE', #56036, .T. ) ;
#107477=EDGE_CURVE ( 'NONE', #15129, #57241, #17319, .T. ) ;
#107478=ORIENTED_EDGE ( 'NONE', *, *, #70900, .F. ) ;
#107479=LINE ( 'NONE', #28277, #122968 ) ;
#107481=ADVANCED_FACE ( 'NONE', ( #16172 ), #38439, .T. ) ;
#107482=DIRECTION ( 'NONE',  ( 0.000000000000000000, 0.000000000000000000, 1.000000000000000000 ) ) ;
#107483=ADVANCED_FACE ( 'NONE', ( #108434 ), #94416, .T. ) ;
#107484=EDGE_CURVE ( 'NONE', #113061, #51178, #79006, .T. ) ;
#107485=DIRECTION ( 'NONE',  ( 0.000000000000000000, -0.9999939076577903929, 0.003490651415223739937 ) ) ;
#107486=CIRCLE ( 'NONE', #46853, 0.06509327318403745899 ) ;
#107487=DIRECTION ( 'NONE',  ( -0.000000000000000000, -1.000000000000000000, -0.000000000000000000 ) ) ;
#107488=ORIENTED_EDGE ( 'NONE', *, *, #102019, .T. ) ;
#107489=ORIENTED_EDGE ( 'NONE', *, *, #32835, .F. ) ;
#107490=CARTESIAN_POINT ( 'NONE',  ( -12.29999999999999716, 2.500000000000000000, 0.4464101615137776591 ) ) ;
#107491=ADVANCED_FACE ( 'NONE', ( #6999 ), #118258, .T. ) ;
#107492=ORIENTED_EDGE ( 'NONE', *, *, #121126, .F. ) ;
#107493=AXIS2_PLACEMENT_3D ( 'NONE', #69221, #477, #29973 ) ;
#107494=FACE_OUTER_BOUND ( 'NONE', #29704, .T. ) ;
#107495=CARTESIAN_POINT ( 'NONE',  ( 12.49999999999990408, 2.500000000000000000, -3.737306695894649700 ) ) ;
#107497=EDGE_LOOP ( 'NONE', ( #103412, #94091, #116278, #28427 ) ) ;
#107499=FACE_OUTER_BOUND ( 'NONE', #21792, .T. ) ;
#107500=CARTESIAN_POINT ( 'NONE',  ( -12.49999999999999289, 12.50000000000000000, -0.7579135962115874925 ) ) ;
#107501=DIRECTION ( 'NONE',  ( 0.000000000000000000, 0.000000000000000000, 1.000000000000000000 ) ) ;
#107502=ORIENTED_EDGE ( 'NONE', *, *, #76362, .T. ) ;
#107503=VECTOR ( 'NONE', #91247, 1000.000000000000000 ) ;
#107504=DIRECTION ( 'NONE',  ( -0.000000000000000000, -1.000000000000000000, -0.000000000000000000 ) ) ;
#107505=CARTESIAN_POINT ( 'NONE',  ( -14.79999999999998295, 2.500000000000000000, -0.2464101615137760659 ) ) ;
#107507=CARTESIAN_POINT ( 'NONE',  ( 4.549999999999935874, 12.50000000000000000, 6.495190528383297135 ) ) ;
#107508=CARTESIAN_POINT ( 'NONE',  ( 10.59999999999990905, 2.500000000000000000, 4.676537180435972552 ) ) ;
#107509=LINE ( 'NONE', #77406, #86747 ) ;
#107510=EDGE_LOOP ( 'NONE', ( #78774, #23587, #71509, #35901 ) ) ;
#107511=AXIS2_PLACEMENT_3D ( 'NONE', #40740, #11239, #51832 ) ;
#107512=AXIS2_PLACEMENT_3D ( 'NONE', #50527, #10588, #122508 ) ;
#107513=DIRECTION ( 'NONE',  ( 0.000000000000000000, -0.9999939076577903929, 0.003490651415223739937 ) ) ;
#107514=AXIS2_PLACEMENT_3D ( 'NONE', #20473, #82622, #30309 ) ;
#107515=EDGE_LOOP ( 'NONE', ( #5821, #121741, #35863, #127401 ) ) ;
#107516=EDGE_CURVE ( 'NONE', #89903, #110245, #6558, .T. ) ;
#107517=DIRECTION ( 'NONE',  ( 0.000000000000000000, 0.000000000000000000, 1.000000000000000000 ) ) ;
#107518=CARTESIAN_POINT ( 'NONE',  ( -7.950000000000012612, 2.500000000000000000, 2.165063509461097713 ) ) ;
#107519=CARTESIAN_POINT ( 'NONE',  ( 9.149999999999916866, 2.500000000000000000, 5.802370205355744659 ) ) ;
#107520=ADVANCED_FACE ( 'NONE', ( #46961 ), #67199, .T. ) ;
#107521=ORIENTED_EDGE ( 'NONE', *, *, #94762, .T. ) ;
#107522=DIRECTION ( 'NONE',  ( 0.000000000000000000, 1.000000000000000000, 0.000000000000000000 ) ) ;
#107523=EDGE_CURVE ( 'NONE', #2500, #120531, #315, .T. ) ;
#107524=FACE_OUTER_BOUND ( 'NONE', #45420, .T. ) ;
#107525=ORIENTED_EDGE ( 'NONE', *, *, #128901, .T. ) ;
#107526=CARTESIAN_POINT ( 'NONE',  ( -0.4000000000000339950, 12.50000000000000000, 0.6928203230275518099 ) ) ;
#107527=EDGE_CURVE ( 'NONE', #74144, #65189, #44240, .T. ) ;
#107528=VERTEX_POINT ( 'NONE', #96044 ) ;
#107529=LINE ( 'NONE', #85934, #70402 ) ;
#107530=EDGE_CURVE ( 'NONE', #269, #84610, #81888, .T. ) ;
#107531=EDGE_CURVE ( 'NONE', #31429, #116085, #11071, .T. ) ;
#107532=CONICAL_SURFACE ( 'NONE', #72041, 0.1000000000000002554, 0.003490658503988666988 ) ;
#107533=ORIENTED_EDGE ( 'NONE', *, *, #111878, .F. ) ;
#107534=CARTESIAN_POINT ( 'NONE',  ( -12.09999999999999609, 12.50000000000000000, -3.702399969078684627 ) ) ;
#107535=CARTESIAN_POINT ( 'NONE',  ( -9.600000000000006750, 2.500000000000000000, 3.537306695894645081 ) ) ;
#107536=VECTOR ( 'NONE', #92000, 1000.000000000000000 ) ;
#107537=EDGE_LOOP ( 'NONE', ( #84960, #78523, #124772, #15750 ) ) ;
#107538=EDGE_LOOP ( 'NONE', ( #47974, #16717 ) ) ;
#107539=CARTESIAN_POINT ( 'NONE',  ( 0.1999999999999567124, 12.50000000000000000, -3.983716857408426293 ) ) ;
#107540=CARTESIAN_POINT ( 'NONE',  ( 8.549999999999920774, 12.50000000000000000, -2.576566944158915184 ) ) ;
#107541=EDGE_LOOP ( 'NONE', ( #71969, #69789, #69208, #94987 ) ) ;
#107542=ADVANCED_FACE ( 'NONE', ( #126152 ), #60974, .T. ) ;
#107543=DIRECTION ( 'NONE',  ( 0.000000000000000000, 0.000000000000000000, 1.000000000000000000 ) ) ;
#107544=DIRECTION ( 'NONE',  ( 0.000000000000000000, 1.000000000000000000, 0.000000000000000000 ) ) ;
#107546=AXIS2_PLACEMENT_3D ( 'NONE', #30800, #119803, #668 ) ;
#107547=VECTOR ( 'NONE', #24541, 1000.000000000000000 ) ;
#107548=DIRECTION ( 'NONE',  ( 0.000000000000000000, 1.000000000000000000, 0.000000000000000000 ) ) ;
#107549=DIRECTION ( 'NONE',  ( 0.000000000000000000, 0.000000000000000000, 1.000000000000000000 ) ) ;
#107550=LINE ( 'NONE', #17866, #95434 ) ;
#107551=DIRECTION ( 'NONE',  ( 0.000000000000000000, 1.000000000000000000, 0.000000000000000000 ) ) ;
#107552=CIRCLE ( 'NONE', #109617, 0.06509327318403741736 ) ;
#107553=VECTOR ( 'NONE', #121076, 1000.000000000000000 ) ;
#107554=EDGE_LOOP ( 'NONE', ( #45757, #63004, #29886, #103860 ) ) ;
#107556=ORIENTED_EDGE ( 'NONE', *, *, #29993, .T. ) ;
#107557=VERTEX_POINT ( 'NONE', #37141 ) ;
#107558=CARTESIAN_POINT ( 'NONE',  ( -10.84999999999999964, 2.500000000000000000, 7.188010851410848723 ) ) ;
#107559=DIRECTION ( 'NONE',  ( 0.000000000000000000, 0.000000000000000000, -1.000000000000000000 ) ) ;
#107560=CIRCLE ( 'NONE', #67844, 0.1000000000000000472 ) ;
#107561=DIRECTION ( 'NONE',  ( 0.000000000000000000, 0.000000000000000000, 1.000000000000000000 ) ) ;
#107562=EDGE_LOOP ( 'NONE', ( #17390, #26389, #109512, #97797 ) ) ;
#107563=FACE_BOUND ( 'NONE', #18366, .T. ) ;
#107564=EDGE_LOOP ( 'NONE', ( #58324, #118942 ) ) ;
#107565=ADVANCED_FACE ( 'NONE', ( #116958 ), #73487, .T. ) ;
#107566=CARTESIAN_POINT ( 'NONE',  ( 4.149999999999941735, 12.50000000000000000, -7.188010851410854052 ) ) ;
#107567=DIRECTION ( 'NONE',  ( 0.000000000000000000, -0.9999939076577903929, 0.003490651415223739937 ) ) ;
#107568=DIRECTION ( 'NONE',  ( 1.000000000000000000, 0.000000000000000000, 0.000000000000000000 ) ) ;
#107569=CARTESIAN_POINT ( 'NONE',  ( -2.500000000000032419, 2.500000000000000000, -3.637306695894650055 ) ) ;
#107570=DIRECTION ( 'NONE',  ( 0.000000000000000000, 0.000000000000000000, -1.000000000000000000 ) ) ;
#107571=CARTESIAN_POINT ( 'NONE',  ( -0.2000000000000408673, 12.50000000000000000, -3.983716857408426293 ) ) ;
#107572=CARTESIAN_POINT ( 'NONE',  ( 2.049999999999950084, 12.50000000000000000, -6.495190528383302464 ) ) ;
#107573=DIRECTION ( 'NONE',  ( 0.000000000000000000, 1.000000000000000000, 0.000000000000000000 ) ) ;
#107574=CARTESIAN_POINT ( 'NONE',  ( 11.24999999999994493, 2.500000000000000000, 6.495190528383297135 ) ) ;
#107575=AXIS2_PLACEMENT_3D ( 'NONE', #84612, #124541, #34888 ) ;
#107576=DIRECTION ( 'NONE',  ( -0.000000000000000000, -1.000000000000000000, -0.000000000000000000 ) ) ;
#107577=ORIENTED_EDGE ( 'NONE', *, *, #9950, .F. ) ;
#107578=ORIENTED_EDGE ( 'NONE', *, *, #103081, .T. ) ;
#107580=VERTEX_POINT ( 'NONE', #89448 ) ;
#107581=ORIENTED_EDGE ( 'NONE', *, *, #31675, .F. ) ;
#107582=CARTESIAN_POINT ( 'NONE',  ( 17.50000000000001066, -2.481874158964551658, -3.264437049507144195 ) ) ;
#107583=CARTESIAN_POINT ( 'NONE',  ( 13.14999999999989733, 2.500000000000000000, -1.818653347947325916 ) ) ;
#107584=EDGE_LOOP ( 'NONE', ( #108704, #83153, #642, #41920 ) ) ;
#107585=ORIENTED_EDGE ( 'NONE', *, *, #70690, .T. ) ;
#107586=VERTEX_POINT ( 'NONE', #52113 ) ;
#107587=DIRECTION ( 'NONE',  ( -4.274815082592931898E-19, -0.9999939076577903929, -0.003490651415223739937 ) ) ;
#107588=CIRCLE ( 'NONE', #15619, 0.1000000000000000472 ) ;
#107589=AXIS2_PLACEMENT_3D ( 'NONE', #77111, #85633, #35895 ) ;
#107590=DIRECTION ( 'NONE',  ( -0.000000000000000000, 1.000000000000000000, -0.000000000000000000 ) ) ;
#107591=CARTESIAN_POINT ( 'NONE',  ( -7.100000000000014744, 2.500000000000000000, 4.230127018922196669 ) ) ;
#107592=LINE ( 'NONE', #27728, #109564 ) ;
#107594=FACE_OUTER_BOUND ( 'NONE', #84058, .T. ) ;
#107595=EDGE_CURVE ( 'NONE', #104575, #99398, #40356, .T. ) ;
#107596=ORIENTED_EDGE ( 'NONE', *, *, #20196, .T. ) ;
#107597=DIRECTION ( 'NONE',  ( 0.000000000000000000, 0.000000000000000000, 1.000000000000000000 ) ) ;
#107598=ORIENTED_EDGE ( 'NONE', *, *, #20125, .T. ) ;
#107599=ORIENTED_EDGE ( 'NONE', *, *, #49877, .T. ) ;
#107600=ORIENTED_EDGE ( 'NONE', *, *, #9682, .T. ) ;
#107601=VECTOR ( 'NONE', #79856, 1000.000000000000000 ) ;
#107602=DIRECTION ( 'NONE',  ( 0.000000000000000000, 0.000000000000000000, 1.000000000000000000 ) ) ;
#107603=ORIENTED_EDGE ( 'NONE', *, *, #45918, .T. ) ;
#107604=VERTEX_POINT ( 'NONE', #80930 ) ;
#107605=DIRECTION ( 'NONE',  ( -0.000000000000000000, 1.000000000000000000, -0.000000000000000000 ) ) ;
#107606=DIRECTION ( 'NONE',  ( -0.000000000000000000, 1.000000000000000000, -0.000000000000000000 ) ) ;
#107607=CIRCLE ( 'NONE', #57433, 0.1000000000000002554 ) ;
#107608=DIRECTION ( 'NONE',  ( 0.000000000000000000, 1.000000000000000000, 0.000000000000000000 ) ) ;
#107609=AXIS2_PLACEMENT_3D ( 'NONE', #114314, #105786, #46215 ) ;
#107610=DIRECTION ( 'NONE',  ( -0.000000000000000000, -1.000000000000000000, -0.000000000000000000 ) ) ;
#107611=CARTESIAN_POINT ( 'NONE',  ( 2.899999999999946620, 12.50000000000000000, -5.022947341949754119 ) ) ;
#107612=AXIS2_PLACEMENT_3D ( 'NONE', #6580, #47200, #97572 ) ;
#107613=VERTEX_POINT ( 'NONE', #129407 ) ;
#107614=VECTOR ( 'NONE', #124104, 1000.000000000000000 ) ;
#107615=PLANE ( 'NONE',  #107643 ) ;
#107616=ORIENTED_EDGE ( 'NONE', *, *, #911, .F. ) ;
#107617=CARTESIAN_POINT ( 'NONE',  ( -3.950000000000026379, 2.500000000000000000, 6.841600689897072485 ) ) ;
#107618=ADVANCED_FACE ( 'NONE', ( #110997 ), #121608, .T. ) ;
#107619=ORIENTED_EDGE ( 'NONE', *, *, #105422, .T. ) ;
#107620=DIRECTION ( 'NONE',  ( -0.000000000000000000, -1.000000000000000000, -0.000000000000000000 ) ) ;
#107621=CARTESIAN_POINT ( 'NONE',  ( -4.800000000000026468, 2.500000000000000000, -4.776537180435978414 ) ) ;
#107622=ORIENTED_EDGE ( 'NONE', *, *, #38031, .F. ) ;
#107623=DIRECTION ( 'NONE',  ( -0.000000000000000000, -1.000000000000000000, -0.000000000000000000 ) ) ;
#107625=ORIENTED_EDGE ( 'NONE', *, *, #32757, .F. ) ;
#107626=AXIS2_PLACEMENT_3D ( 'NONE', #107294, #117740, #88275 ) ;
#107627=VECTOR ( 'NONE', #12152, 1000.000000000000000 ) ;
#107628=DIRECTION ( 'NONE',  ( 0.000000000000000000, 1.000000000000000000, 0.000000000000000000 ) ) ;
#107629=VERTEX_POINT ( 'NONE', #41664 ) ;
#107630=CIRCLE ( 'NONE', #103429, 0.06509327318403745899 ) ;
#107631=EDGE_CURVE ( 'NONE', #91861, #107707, #109741, .T. ) ;
#107632=AXIS2_PLACEMENT_3D ( 'NONE', #109006, #126740, #99217 ) ;
#107633=EDGE_CURVE ( 'NONE', #50900, #116451, #79627, .T. ) ;
#107634=EDGE_LOOP ( 'NONE', ( #32667, #42260 ) ) ;
#107635=CARTESIAN_POINT ( 'NONE',  ( -5.200000000000020606, 2.500000000000000000, 3.983716857408420964 ) ) ;
#107637=EDGE_CURVE ( 'NONE', #55845, #124238, #21262, .T. ) ;
#107640=FACE_OUTER_BOUND ( 'NONE', #79475, .T. ) ;
#107641=CARTESIAN_POINT ( 'NONE',  ( 13.94999999999989448, 2.500000000000000000, -2.511473670974877948 ) ) ;
#107642=CIRCLE ( 'NONE', #11491, 0.06509327318403743123 ) ;
#107643=AXIS2_PLACEMENT_3D ( 'NONE', #97791, #8114, #108882 ) ;
#107644=ADVANCED_FACE ( 'NONE', ( #29887 ), #39734, .T. ) ;
#107645=CARTESIAN_POINT ( 'NONE',  ( -9.400000000000009237, 12.50000000000000000, -4.741630453620011565 ) ) ;
#107646=AXIS2_PLACEMENT_3D ( 'NONE', #18129, #7009, #127456 ) ;
#107647=ADVANCED_FACE ( 'NONE', ( #71097 ), #100675, .T. ) ;
#107648=ORIENTED_EDGE ( 'NONE', *, *, #97448, .F. ) ;
#107649=EDGE_CURVE ( 'NONE', #48724, #54992, #31741, .T. ) ;
#107650=AXIS2_PLACEMENT_3D ( 'NONE', #115657, #16152, #83006 ) ;
#107651=DIRECTION ( 'NONE',  ( 0.000000000000000000, 0.000000000000000000, 1.000000000000000000 ) ) ;
#107652=DIRECTION ( 'NONE',  ( 0.000000000000000000, -0.9999939076577903929, 0.003490651415223739937 ) ) ;
#107653=CIRCLE ( 'NONE', #76351, 0.06509327318403741736 ) ;
#107655=ORIENTED_EDGE ( 'NONE', *, *, #98833, .F. ) ;
#107656=CONICAL_SURFACE ( 'NONE', #114007, 0.1000000000000002554, 0.003490658503988666988 ) ;
#107657=CARTESIAN_POINT ( 'NONE',  ( 8.349999999999923261, 2.500000000000000000, -5.802370205355749988 ) ) ;
#107658=CARTESIAN_POINT ( 'NONE',  ( 9.999999999999911182, 2.500000000000000000, 5.022947341949748790 ) ) ;
#107659=CARTESIAN_POINT ( 'NONE',  ( -6.071532165918824830E-15, 12.50000000000000000, -4.330127018922201643 ) ) ;
#107660=CARTESIAN_POINT ( 'NONE',  ( 14.99999999999989164, 12.50000000000000000, 0.6928203230275494784 ) ) ;
#107661=EDGE_CURVE ( 'NONE', #110789, #71913, #71424, .T. ) ;
#107662=CARTESIAN_POINT ( 'NONE',  ( 15.39999999999989022, 12.50000000000000000, -2.385244779468109755E-15 ) ) ;
#107663=EDGE_LOOP ( 'NONE', ( #1, #3026, #11251, #6970 ) ) ;
#107664=DIRECTION ( 'NONE',  ( -0.000000000000000000, -1.000000000000000000, -0.000000000000000000 ) ) ;
#107665=DIRECTION ( 'NONE',  ( 0.000000000000000000, 0.000000000000000000, 1.000000000000000000 ) ) ;
#107666=AXIS2_PLACEMENT_3D ( 'NONE', #80685, #30307, #29639 ) ;
#107667=VERTEX_POINT ( 'NONE', #90075 ) ;
#107668=PLANE ( 'NONE',  #28087 ) ;
#107669=VERTEX_POINT ( 'NONE', #71751 ) ;
#107670=EDGE_LOOP ( 'NONE', ( #113901, #125382, #76094, #94321 ) ) ;
#107671=DIRECTION ( 'NONE',  ( 0.000000000000000000, -0.9999939076577903929, 0.003490651415223739937 ) ) ;
#107672=ORIENTED_EDGE ( 'NONE', *, *, #2136, .F. ) ;
#107673=FACE_OUTER_BOUND ( 'NONE', #112889, .T. ) ;
#107675=CIRCLE ( 'NONE', #88893, 0.1000000000000000472 ) ;
#107676=DIRECTION ( 'NONE',  ( 0.000000000000000000, 0.000000000000000000, 1.000000000000000000 ) ) ;
#107677=AXIS2_PLACEMENT_3D ( 'NONE', #23991, #41074, #42345 ) ;
#107678=VERTEX_POINT ( 'NONE', #60016 ) ;
#107679=CARTESIAN_POINT ( 'NONE',  ( -4.150000000000024336, 2.500000000000000000, 1.572243186433545548 ) ) ;
#107680=DIRECTION ( 'NONE',  ( -0.000000000000000000, 1.000000000000000000, -0.000000000000000000 ) ) ;
#107681=ORIENTED_EDGE ( 'NONE', *, *, #13016, .T. ) ;
#107682=PLANE ( 'NONE',  #4696 ) ;
#107683=CARTESIAN_POINT ( 'NONE',  ( 10.44999999999991047, 12.50000000000000000, 2.099970236277060032 ) ) ;
#107684=ORIENTED_EDGE ( 'NONE', *, *, #88118, .T. ) ;
#107685=CIRCLE ( 'NONE', #74238, 0.06509327318403745899 ) ;
#107686=ADVANCED_FACE ( 'NONE', ( #111675 ), #40057, .T. ) ;
#107687=ORIENTED_EDGE ( 'NONE', *, *, #47864, .T. ) ;
#107688=CONICAL_SURFACE ( 'NONE', #34556, 0.1000000000000002554, 0.003490658503988666988 ) ;
#107689=ADVANCED_FACE ( 'NONE', ( #40366 ), #48457, .T. ) ;
#107690=ORIENTED_EDGE ( 'NONE', *, *, #52723, .T. ) ;
#107691=CARTESIAN_POINT ( 'NONE',  ( 11.69999999999990870, 12.50000000000000000, -4.330127018922201643 ) ) ;
#107692=DIRECTION ( 'NONE',  ( 0.000000000000000000, -0.000000000000000000, 1.000000000000000000 ) ) ;
#107693=CARTESIAN_POINT ( 'NONE',  ( -12.49999999999999289, 12.50000000000000000, 3.637306695894644726 ) ) ;
#107694=FACE_BOUND ( 'NONE', #9056, .T. ) ;
#107695=ORIENTED_EDGE ( 'NONE', *, *, #15056, .F. ) ;
#107696=DIRECTION ( 'NONE',  ( 0.000000000000000000, 0.000000000000000000, 1.000000000000000000 ) ) ;
#107697=DIRECTION ( 'NONE',  ( 0.000000000000000000, 1.000000000000000000, 0.000000000000000000 ) ) ;
#107698=ORIENTED_EDGE ( 'NONE', *, *, #85232, .F. ) ;
#107699=EDGE_CURVE ( 'NONE', #104854, #113368, #107229, .T. ) ;
#107700=AXIS2_PLACEMENT_3D ( 'NONE', #105767, #46854, #37678 ) ;
#107702=AXIS2_PLACEMENT_3D ( 'NONE', #24495, #126567, #123970 ) ;
#107703=CARTESIAN_POINT ( 'NONE',  ( -6.250000000000017764, 12.50000000000000000, 7.188010851410848723 ) ) ;
#107704=CARTESIAN_POINT ( 'NONE',  ( 12.09999999999990550, 12.50000000000000000, -4.330127018922201643 ) ) ;
#107705=CARTESIAN_POINT ( 'NONE',  ( -1.650000000000035660, 2.500000000000000000, 7.188010851410848723 ) ) ;
#107706=CARTESIAN_POINT ( 'NONE',  ( 4.149999999999939959, 2.500000000000000000, -6.495190528383302464 ) ) ;
#107707=VERTEX_POINT ( 'NONE', #66903 ) ;
#107708=ORIENTED_EDGE ( 'NONE', *, *, #72304, .F. ) ;
#107709=ORIENTED_EDGE ( 'NONE', *, *, #19775, .T. ) ;
#107710=VERTEX_POINT ( 'NONE', #96357 ) ;
#107711=ORIENTED_EDGE ( 'NONE', *, *, #64064, .T. ) ;
#107712=CARTESIAN_POINT ( 'NONE',  ( 2.699999999999946443, 12.50000000000000000, -3.918623584224389056 ) ) ;
#107713=DIRECTION ( 'NONE',  ( 0.000000000000000000, -0.9999939076577903929, 0.003490651415223739937 ) ) ;
#107714=ORIENTED_EDGE ( 'NONE', *, *, #24902, .F. ) ;
#107715=FACE_BOUND ( 'NONE', #23068, .T. ) ;
#107716=AXIS2_PLACEMENT_3D ( 'NONE', #64130, #85701, #24857 ) ;
#107717=CARTESIAN_POINT ( 'NONE',  ( 6.899999999999928413, 2.500000000000000000, -4.676537180435977881 ) ) ;
#107718=AXIS2_PLACEMENT_3D ( 'NONE', #44351, #12945, #101998 ) ;
#107719=CARTESIAN_POINT ( 'NONE',  ( -13.14999999999999147, 12.50000000000000000, 1.818653347947325472 ) ) ;
#107720=DIRECTION ( 'NONE',  ( -0.000000000000000000, -1.000000000000000000, -0.000000000000000000 ) ) ;
#107721=CARTESIAN_POINT ( 'NONE',  ( 4.349999999999941025, 2.500000000000000000, -1.818653347947326138 ) ) ;
#107722=DIRECTION ( 'NONE',  ( 0.000000000000000000, 0.000000000000000000, 1.000000000000000000 ) ) ;
#107723=VERTEX_POINT ( 'NONE', #42963 ) ;
#107724=DIRECTION ( 'NONE',  ( 0.000000000000000000, 1.000000000000000000, 0.000000000000000000 ) ) ;
#107725=CIRCLE ( 'NONE', #13711, 0.09999999999999982514 ) ;
#107726=EDGE_LOOP ( 'NONE', ( #109487, #70237, #19942, #114762 ) ) ;
#107727=CIRCLE ( 'NONE', #5305, 0.06509327318403745899 ) ;
#107728=AXIS2_PLACEMENT_3D ( 'NONE', #123864, #53853, #65597 ) ;
#107729=EDGE_LOOP ( 'NONE', ( #87667, #93831 ) ) ;
#107730=ORIENTED_EDGE ( 'NONE', *, *, #93601, .F. ) ;
#107731=LINE ( 'NONE', #88734, #104891 ) ;
#107732=CARTESIAN_POINT ( 'NONE',  ( -8.550000000000013145, 12.50000000000000000, 2.511473670974873507 ) ) ;
#107733=CARTESIAN_POINT ( 'NONE',  ( 15.39999999999989022, 12.50000000000000000, -0.06509327318403980434 ) ) ;
#107734=ORIENTED_EDGE ( 'NONE', *, *, #87974, .T. ) ;
#107735=DIRECTION ( 'NONE',  ( 0.000000000000000000, 0.000000000000000000, 1.000000000000000000 ) ) ;
#107736=AXIS2_PLACEMENT_3D ( 'NONE', #5553, #34407, #55318 ) ;
#107737=CARTESIAN_POINT ( 'NONE',  ( 11.64999999999990621, 12.50000000000000000, 6.495190528383297135 ) ) ;
#107738=CARTESIAN_POINT ( 'NONE',  ( -11.64999999999999680, 2.500000000000000000, 5.902370205355745192 ) ) ;
#107739=DIRECTION ( 'NONE',  ( 0.000000000000000000, 0.000000000000000000, -1.000000000000000000 ) ) ;
#107740=CARTESIAN_POINT ( 'NONE',  ( 1.249999999999952482, 2.500000000000000000, -5.802370205355749988 ) ) ;
#107741=LINE ( 'NONE', #39037, #88521 ) ;
#107742=AXIS2_PLACEMENT_3D ( 'NONE', #61612, #89764, #22333 ) ;
#107743=ADVANCED_FACE ( 'NONE', ( #7338 ), #21358, .T. ) ;
#107744=CARTESIAN_POINT ( 'NONE',  ( -6.050000000000017586, 12.50000000000000000, 6.148780366869520009 ) ) ;
#107745=ADVANCED_FACE ( 'NONE', ( #14095 ), #116012, .T. ) ;
#107746=VERTEX_POINT ( 'NONE', #62581 ) ;
#107747=CARTESIAN_POINT ( 'NONE',  ( -7.500000000000001776, -2.500000000000000000, 9.000000000000003553 ) ) ;
#107748=ORIENTED_EDGE ( 'NONE', *, *, #13602, .F. ) ;
#107749=ORIENTED_EDGE ( 'NONE', *, *, #11419, .T. ) ;
#107750=DIRECTION ( 'NONE',  ( 0.000000000000000000, 1.000000000000000000, 0.000000000000000000 ) ) ;
#107751=DIRECTION ( 'NONE',  ( 0.000000000000000000, 0.000000000000000000, 1.000000000000000000 ) ) ;
#107752=DIRECTION ( 'NONE',  ( -0.000000000000000000, 1.000000000000000000, -0.000000000000000000 ) ) ;
#107753=EDGE_CURVE ( 'NONE', #64553, #83521, #69377, .T. ) ;
#107754=AXIS2_PLACEMENT_3D ( 'NONE', #14483, #23684, #73418 ) ;
#107755=ORIENTED_EDGE ( 'NONE', *, *, #117977, .T. ) ;
#107756=EDGE_LOOP ( 'NONE', ( #437, #43521, #84619, #81792 ) ) ;
#107757=DIRECTION ( 'NONE',  ( 0.000000000000000000, 0.000000000000000000, -1.000000000000000000 ) ) ;
#107758=FACE_OUTER_BOUND ( 'NONE', #43673, .T. ) ;
#107759=DIRECTION ( 'NONE',  ( -0.000000000000000000, 1.000000000000000000, -0.000000000000000000 ) ) ;
#107760=ORIENTED_EDGE ( 'NONE', *, *, #111780, .F. ) ;
#107761=ORIENTED_EDGE ( 'NONE', *, *, #61385, .T. ) ;
#107762=CARTESIAN_POINT ( 'NONE',  ( -4.350000000000023626, 2.500000000000000000, -1.918653347947325782 ) ) ;
#107763=AXIS2_PLACEMENT_3D ( 'NONE', #53161, #121889, #80691 ) ;
#107764=ORIENTED_EDGE ( 'NONE', *, *, #107368, .F. ) ;
#107765=CARTESIAN_POINT ( 'NONE',  ( -3.550000000000030909, 2.500000000000000000, -6.841600689897078702 ) ) ;
#107766=CIRCLE ( 'NONE', #105624, 0.1000000000000000472 ) ;
#107767=FACE_OUTER_BOUND ( 'NONE', #106202, .T. ) ;
#107768=ORIENTED_EDGE ( 'NONE', *, *, #13621, .T. ) ;
#107769=DIRECTION ( 'NONE',  ( 0.000000000000000000, 1.000000000000000000, 0.000000000000000000 ) ) ;
#107770=EDGE_CURVE ( 'NONE', #61867, #30241, #44341, .T. ) ;
#107771=DIRECTION ( 'NONE',  ( 0.000000000000000000, 1.000000000000000000, 0.000000000000000000 ) ) ;
#107772=LINE ( 'NONE', #10833, #57363 ) ;
#107773=DIRECTION ( 'NONE',  ( 0.000000000000000000, -0.000000000000000000, 1.000000000000000000 ) ) ;
#107774=VERTEX_POINT ( 'NONE', #17132 ) ;
#107775=CIRCLE ( 'NONE', #97316, 0.1000000000000000056 ) ;
#107776=EDGE_CURVE ( 'NONE', #97390, #65136, #96553, .T. ) ;
#107777=CARTESIAN_POINT ( 'NONE',  ( -10.85000000000000142, 12.50000000000000000, 2.165063509461097713 ) ) ;
#107778=AXIS2_PLACEMENT_3D ( 'NONE', #94673, #15460, #86122 ) ;
#107779=ORIENTED_EDGE ( 'NONE', *, *, #35261, .T. ) ;
#107780=VERTEX_POINT ( 'NONE', #6672 ) ;
#107781=ADVANCED_FACE ( 'NONE', ( #57090 ), #97019, .T. ) ;
#107782=EDGE_CURVE ( 'NONE', #124302, #59948, #19193, .T. ) ;
#107783=DIRECTION ( 'NONE',  ( 0.000000000000000000, 0.000000000000000000, -1.000000000000000000 ) ) ;
#107784=DIRECTION ( 'NONE',  ( -0.000000000000000000, 1.000000000000000000, -0.000000000000000000 ) ) ;
#107785=LINE ( 'NONE', #116941, #13383 ) ;
#107786=ADVANCED_FACE ( 'NONE', ( #46000 ), #12798, .T. ) ;
#107787=DIRECTION ( 'NONE',  ( -0.000000000000000000, -1.000000000000000000, -0.000000000000000000 ) ) ;
#107788=EDGE_CURVE ( 'NONE', #24991, #75374, #25543, .T. ) ;
#107789=CARTESIAN_POINT ( 'NONE',  ( -3.350000000000028511, 12.50000000000000000, 1.407149913249508000 ) ) ;
#107790=DIRECTION ( 'NONE',  ( 0.000000000000000000, 1.000000000000000000, 0.000000000000000000 ) ) ;
#107791=AXIS2_PLACEMENT_3D ( 'NONE', #76799, #104942, #114773 ) ;
#107792=LINE ( 'NONE', #117579, #75954 ) ;
#107793=DIRECTION ( 'NONE',  ( 0.000000000000000000, 1.000000000000000000, 0.000000000000000000 ) ) ;
#107795=EDGE_CURVE ( 'NONE', #97087, #41669, #72400, .T. ) ;
#107796=EDGE_CURVE ( 'NONE', #5168, #100174, #93322, .T. ) ;
#107797=DIRECTION ( 'NONE',  ( 0.000000000000000000, 0.000000000000000000, 1.000000000000000000 ) ) ;
#107798=ADVANCED_FACE ( 'NONE', ( #36826 ), #126491, .T. ) ;
#107799=EDGE_CURVE ( 'NONE', #96322, #54140, #98706, .T. ) ;
#107800=VERTEX_POINT ( 'NONE', #53401 ) ;
#107801=DIRECTION ( 'NONE',  ( 0.000000000000000000, 0.000000000000000000, -1.000000000000000000 ) ) ;
#107802=DIRECTION ( 'NONE',  ( -0.000000000000000000, -1.000000000000000000, -0.000000000000000000 ) ) ;
#107803=LINE ( 'NONE', #88804, #57937 ) ;
#107804=CARTESIAN_POINT ( 'NONE',  ( 13.09999999999990195, 12.50000000000000000, 3.983716857408420076 ) ) ;
#107805=CARTESIAN_POINT ( 'NONE',  ( -1.900000000000035438, 12.50000000000000000, 3.983716857408420076 ) ) ;
#107806=EDGE_CURVE ( 'NONE', #44808, #81692, #100760, .T. ) ;
#107807=VERTEX_POINT ( 'NONE', #63859 ) ;
#107808=DIRECTION ( 'NONE',  ( 0.000000000000000000, 0.000000000000000000, -1.000000000000000000 ) ) ;
#107809=VECTOR ( 'NONE', #25131, 1000.000000000000000 ) ;
#107810=VECTOR ( 'NONE', #51949, 1000.000000000000000 ) ;
#107811=DIRECTION ( 'NONE',  ( 0.000000000000000000, 1.000000000000000000, 0.000000000000000000 ) ) ;
#107812=CARTESIAN_POINT ( 'NONE',  ( 3.949999999999938005, 12.50000000000000000, 6.841600689897072485 ) ) ;
#107813=ORIENTED_EDGE ( 'NONE', *, *, #95206, .F. ) ;
#107814=ORIENTED_EDGE ( 'NONE', *, *, #56087, .T. ) ;
#107815=VERTEX_POINT ( 'NONE', #103783 ) ;
#107816=ORIENTED_EDGE ( 'NONE', *, *, #102582, .F. ) ;
#107817=VERTEX_POINT ( 'NONE', #76096 ) ;
#107818=CARTESIAN_POINT ( 'NONE',  ( -5.400000000000023448, 2.500000000000000000, -4.230127018922201998 ) ) ;
#107819=CONICAL_SURFACE ( 'NONE', #51416, 0.09999999999999982514, 0.003490658503988666988 ) ;
#107820=EDGE_CURVE ( 'NONE', #60288, #9509, #106204, .T. ) ;
#107821=DIRECTION ( 'NONE',  ( -4.274815082592931898E-19, -0.9999939076577903929, -0.003490651415223739937 ) ) ;
#107822=DIRECTION ( 'NONE',  ( -0.000000000000000000, -1.000000000000000000, -0.000000000000000000 ) ) ;
#107823=AXIS2_PLACEMENT_3D ( 'NONE', #57905, #28437, #57243 ) ;
#107824=DIRECTION ( 'NONE',  ( 0.000000000000000000, 1.000000000000000000, 0.000000000000000000 ) ) ;
#107825=AXIS2_PLACEMENT_3D ( 'NONE', #58325, #68115, #120450 ) ;
#107826=ORIENTED_EDGE ( 'NONE', *, *, #94034, .F. ) ;
#107827=CIRCLE ( 'NONE', #11682, 0.06509327318403743123 ) ;
#107828=CARTESIAN_POINT ( 'NONE',  ( -9.350000000000004974, 12.50000000000000000, 6.776507416713035248 ) ) ;
#107829=AXIS2_PLACEMENT_3D ( 'NONE', #79791, #99450, #121007 ) ;
#107830=EDGE_LOOP ( 'NONE', ( #74040, #23107, #44163, #60709 ) ) ;
#107831=FACE_OUTER_BOUND ( 'NONE', #30776, .T. ) ;
#107832=DIRECTION ( 'NONE',  ( -0.000000000000000000, -1.000000000000000000, -0.000000000000000000 ) ) ;
#107834=DIRECTION ( 'NONE',  ( 0.000000000000000000, 0.000000000000000000, 1.000000000000000000 ) ) ;
#107835=ORIENTED_EDGE ( 'NONE', *, *, #121124, .F. ) ;
#107836=ADVANCED_FACE ( 'NONE', ( #123406 ), #14091, .T. ) ;
#107837=VERTEX_POINT ( 'NONE', #12795 ) ;
#107838=EDGE_LOOP ( 'NONE', ( #81874, #60415, #100421, #32812 ) ) ;
#107839=ADVANCED_FACE ( 'NONE', ( #54035 ), #93959, .T. ) ;
#107840=VERTEX_POINT ( 'NONE', #55330 ) ;
#107841=CARTESIAN_POINT ( 'NONE',  ( 11.84999999999990372, 12.50000000000000000, -6.083687093685488989 ) ) ;
#107842=FACE_OUTER_BOUND ( 'NONE', #88051, .T. ) ;
#107843=CARTESIAN_POINT ( 'NONE',  ( -3.150000000000030553, 2.500000000000000000, 6.148780366869520009 ) ) ;
#107844=FACE_BOUND ( 'NONE', #102424, .T. ) ;
#107845=CARTESIAN_POINT ( 'NONE',  ( -9.550000000000006040, 12.50000000000000000, 2.165063509461097713 ) ) ;
#107846=AXIS2_PLACEMENT_3D ( 'NONE', #68755, #14, #18999 ) ;
#107848=DIRECTION ( 'NONE',  ( 0.000000000000000000, 0.000000000000000000, -1.000000000000000000 ) ) ;
#107849=DIRECTION ( 'NONE',  ( -4.274815082592931898E-19, -0.9999939076577903929, -0.003490651415223739937 ) ) ;
#107851=AXIS2_PLACEMENT_3D ( 'NONE', #37389, #78611, #67447 ) ;
#107852=DIRECTION ( 'NONE',  ( 0.000000000000000000, 1.000000000000000000, 0.000000000000000000 ) ) ;
#107853=DIRECTION ( 'NONE',  ( 0.000000000000000000, 0.000000000000000000, -1.000000000000000000 ) ) ;
#107854=CIRCLE ( 'NONE', #57695, 0.09999999999999982514 ) ;
#107855=CIRCLE ( 'NONE', #120387, 0.06509327318403745899 ) ;
#107856=DIRECTION ( 'NONE',  ( 0.000000000000000000, 1.000000000000000000, 0.000000000000000000 ) ) ;
#107857=ORIENTED_EDGE ( 'NONE', *, *, #97021, .F. ) ;
#107858=EDGE_LOOP ( 'NONE', ( #93495, #61488 ) ) ;
#107859=VERTEX_POINT ( 'NONE', #102491 ) ;
#107860=ORIENTED_EDGE ( 'NONE', *, *, #5049, .F. ) ;
#107861=FACE_OUTER_BOUND ( 'NONE', #124583, .T. ) ;
#107862=FACE_BOUND ( 'NONE', #8500, .T. ) ;
#107863=AXIS2_PLACEMENT_3D ( 'NONE', #96091, #46339, #116366 ) ;
#107864=CARTESIAN_POINT ( 'NONE',  ( -6.050000000000020250, 2.500000000000000000, -6.841600689897078702 ) ) ;
#107866=CIRCLE ( 'NONE', #112084, 0.1000000000000002554 ) ;
#107867=EDGE_LOOP ( 'NONE', ( #15555, #55151 ) ) ;
#107868=LINE ( 'NONE', #27356, #2808 ) ;
#107869=DIRECTION ( 'NONE',  ( 0.000000000000000000, 0.000000000000000000, 1.000000000000000000 ) ) ;
#107870=LINE ( 'NONE', #53144, #87098 ) ;
#107871=ORIENTED_EDGE ( 'NONE', *, *, #66857, .T. ) ;
#107872=CARTESIAN_POINT ( 'NONE',  ( 16.55763163376620284, -0.1615157349257290431, 6.093150851882368713 ) ) ;
#107873=CARTESIAN_POINT ( 'NONE',  ( 21.23528140090977345, 2.699413673072321718, -2.293764360948945757 ) ) ;
#107874=EDGE_CURVE ( 'NONE', #105467, #58293, #27601, .T. ) ;
#107875=VERTEX_POINT ( 'NONE', #105048 ) ;
#107876=EDGE_LOOP ( 'NONE', ( #41269, #9424 ) ) ;
#107877=DIRECTION ( 'NONE',  ( -0.000000000000000000, 1.000000000000000000, -0.000000000000000000 ) ) ;
#107878=CARTESIAN_POINT ( 'NONE',  ( -2.100000000000034284, 12.50000000000000000, -2.385244779468109755E-15 ) ) ;
#107879=CARTESIAN_POINT ( 'NONE',  ( 4.349999999999937472, 12.50000000000000000, 6.841600689897072485 ) ) ;
#107880=DIRECTION ( 'NONE',  ( 0.000000000000000000, 1.000000000000000000, 0.000000000000000000 ) ) ;
#107881=EDGE_LOOP ( 'NONE', ( #100468, #52974 ) ) ;
#107882=DIRECTION ( 'NONE',  ( 0.000000000000000000, 0.000000000000000000, -1.000000000000000000 ) ) ;
#107883=EDGE_LOOP ( 'NONE', ( #74297, #30018 ) ) ;
#107884=ADVANCED_FACE ( 'NONE', ( #3007 ), #56838, .T. ) ;
#107885=EDGE_LOOP ( 'NONE', ( #87957, #3640, #68729, #62643 ) ) ;
#107886=EDGE_CURVE ( 'NONE', #7603, #112348, #2555, .T. ) ;
#107887=DIRECTION ( 'NONE',  ( 0.000000000000000000, 0.000000000000000000, -1.000000000000000000 ) ) ;
#107888=B_SPLINE_CURVE_WITH_KNOTS ( 'NONE', 3,
 ( #52774, #70484, #92709, #3677, #43623, #30585, #50854, #20744, #60684, #100577 ),
 .UNSPECIFIED., .F., .F.,
 ( 4, 2, 2, 2, 4 ),
 ( 4.358438792651350852E-18, 0.0006221151217586977583, 0.001244230243517391180, 0.001866345365276084710, 0.002488460487034778023 ),
 .UNSPECIFIED. ) ;
#107889=ORIENTED_EDGE ( 'NONE', *, *, #19097, .F. ) ;
#107891=FACE_BOUND ( 'NONE', #42611, .T. ) ;
#107892=AXIS2_PLACEMENT_3D ( 'NONE', #15143, #53177, #55101 ) ;
#107893=VERTEX_POINT ( 'NONE', #62578 ) ;
#107894=CIRCLE ( 'NONE', #72407, 0.09999999999999982514 ) ;
#107896=VERTEX_POINT ( 'NONE', #84124 ) ;
#107897=CARTESIAN_POINT ( 'NONE',  ( -6.450000000000016165, 2.500000000000000000, 6.941600689897073018 ) ) ;
#107898=DIRECTION ( 'NONE',  ( 0.000000000000000000, 0.000000000000000000, 1.000000000000000000 ) ) ;
#107899=( BOUNDED_CURVE ( )  B_SPLINE_CURVE ( 2, ( #69321, #77228, #119720 ),
 .UNSPECIFIED., .F., .F. ) 
 B_SPLINE_CURVE_WITH_KNOTS ( ( 3, 3 ),
 ( -5.999999999966287552E-08, 0.01488647113978520606 ),
 .UNSPECIFIED. ) 
 CURVE ( )  GEOMETRIC_REPRESENTATION_ITEM ( )  RATIONAL_B_SPLINE_CURVE ( ( 1.000000000000000000, 0.7762344340431585055, 0.8943752373141855561 ) ) 
 REPRESENTATION_ITEM ( '' )  );
#107900=CARTESIAN_POINT ( 'NONE',  ( 5.649999999999934630, 2.500000000000000000, -2.511473670974877948 ) ) ;
#107902=EDGE_CURVE ( 'NONE', #101722, #53584, #52737, .T. ) ;
#107903=FACE_OUTER_BOUND ( 'NONE', #98913, .T. ) ;
#107904=ORIENTED_EDGE ( 'NONE', *, *, #20081, .T. ) ;
#107905=AXIS2_PLACEMENT_3D ( 'NONE', #121328, #62432, #39585 ) ;
#107906=AXIS2_PLACEMENT_3D ( 'NONE', #6398, #128149, #78425 ) ;
#107907=VERTEX_POINT ( 'NONE', #95257 ) ;
#107908=EDGE_LOOP ( 'NONE', ( #91069, #7497, #103721, #11424 ) ) ;
#107909=CARTESIAN_POINT ( 'NONE',  ( -6.650000000000015454, 12.50000000000000000, 2.922977105672686982 ) ) ;
#107910=DIRECTION ( 'NONE',  ( -0.000000000000000000, 1.000000000000000000, -0.000000000000000000 ) ) ;
#107911=LINE ( 'NONE', #109189, #20858 ) ;
#107913=ORIENTED_EDGE ( 'NONE', *, *, #23284, .F. ) ;
#107914=VERTEX_POINT ( 'NONE', #84782 ) ;
#107915=DIRECTION ( 'NONE',  ( 0.000000000000000000, 1.000000000000000000, 0.000000000000000000 ) ) ;
#107916=CIRCLE ( 'NONE', #66144, 0.1000000000000000056 ) ;
#107917=DIRECTION ( 'NONE',  ( -0.000000000000000000, -1.000000000000000000, -0.000000000000000000 ) ) ;
#107918=CONICAL_SURFACE ( 'NONE', #118288, 0.1000000000000000472, 0.003490658503988666988 ) ;
#107920=CARTESIAN_POINT ( 'NONE',  ( 7.699999999999923794, 12.50000000000000000, -3.983716857408426293 ) ) ;
#107921=DIRECTION ( 'NONE',  ( 0.000000000000000000, 1.000000000000000000, 0.000000000000000000 ) ) ;
#107922=DIRECTION ( 'NONE',  ( 0.000000000000000000, 0.000000000000000000, -1.000000000000000000 ) ) ;
#107923=CARTESIAN_POINT ( 'NONE',  ( -9.150000000000005684, 2.500000000000000000, 6.495190528383297135 ) ) ;
#107924=DIRECTION ( 'NONE',  ( 0.000000000000000000, 0.000000000000000000, -1.000000000000000000 ) ) ;
#107925=DIRECTION ( 'NONE',  ( -0.000000000000000000, -1.000000000000000000, -0.000000000000000000 ) ) ;
#107926=ORIENTED_EDGE ( 'NONE', *, *, #84105, .T. ) ;
#107927=VERTEX_POINT ( 'NONE', #83507 ) ;
#107928=ADVANCED_FACE ( 'NONE', ( #114241 ), #104418, .T. ) ;
#107929=PLANE ( 'NONE',  #71718 ) ;
#107930=CARTESIAN_POINT ( 'NONE',  ( 4.599999999999937472, 12.50000000000000000, 0.6928203230275494784 ) ) ;
#107931=ORIENTED_EDGE ( 'NONE', *, *, #34204, .F. ) ;
#107932=ORIENTED_EDGE ( 'NONE', *, *, #101700, .T. ) ;
#107933=EDGE_CURVE ( 'NONE', #81561, #29893, #61073, .T. ) ;
#107935=DIRECTION ( 'NONE',  ( 0.000000000000000000, 1.000000000000000000, 0.000000000000000000 ) ) ;
#107936=AXIS2_PLACEMENT_3D ( 'NONE', #90827, #11619, #62672 ) ;
#107937=DIRECTION ( 'NONE',  ( -0.000000000000000000, 1.000000000000000000, -0.000000000000000000 ) ) ;
#107938=ADVANCED_FACE ( 'NONE', ( #24571 ), #92359, .T. ) ;
#107939=CARTESIAN_POINT ( 'NONE',  ( -7.500000000000016875, 2.500000000000000000, -3.637306695894650055 ) ) ;
#107940=CARTESIAN_POINT ( 'NONE',  ( -7.100000000000017408, 2.500000000000000000, 0.5928203230275495006 ) ) ;
#107941=DIRECTION ( 'NONE',  ( -0.000000000000000000, 1.000000000000000000, -0.000000000000000000 ) ) ;
#107942=CIRCLE ( 'NONE', #97563, 0.1000000000000000472 ) ;
#107943=CIRCLE ( 'NONE', #80769, 0.1000000000000002554 ) ;
#107944=CARTESIAN_POINT ( 'NONE',  ( 6.899999999999928413, 2.500000000000000000, 4.083716857408421497 ) ) ;
#107945=EDGE_LOOP ( 'NONE', ( #22029, #97595 ) ) ;
#107946=LINE ( 'NONE', #98757, #72803 ) ;
#107947=EDGE_CURVE ( 'NONE', #32914, #86614, #411, .T. ) ;
#107948=EDGE_CURVE ( 'NONE', #72026, #21011, #34417, .T. ) ;
#107949=EDGE_CURVE ( 'NONE', #18418, #118169, #125804, .T. ) ;
#107950=AXIS2_PLACEMENT_3D ( 'NONE', #31566, #71473, #32231 ) ;
#107951=ADVANCED_FACE ( 'NONE', ( #53398 ), #4598, .T. ) ;
#107952=CONICAL_SURFACE ( 'NONE', #72450, 0.09999999999999982514, 0.003490658503988666988 ) ;
#107953=DIRECTION ( 'NONE',  ( 0.000000000000000000, 1.000000000000000000, 0.000000000000000000 ) ) ;
#107954=EDGE_LOOP ( 'NONE', ( #62402, #98273 ) ) ;
#107955=AXIS2_PLACEMENT_3D ( 'NONE', #57487, #26731, #106567 ) ;
#107956=EDGE_CURVE ( 'NONE', #71603, #48770, #79846, .T. ) ;
#107957=VERTEX_POINT ( 'NONE', #25202 ) ;
#107958=ORIENTED_EDGE ( 'NONE', *, *, #126689, .F. ) ;
#107959=EDGE_LOOP ( 'NONE', ( #48526, #79612 ) ) ;
#107960=CARTESIAN_POINT ( 'NONE',  ( 4.399999999999939071, 12.50000000000000000, -0.4115034346978156399 ) ) ;
#107961=DIRECTION ( 'NONE',  ( -4.274815082592931898E-19, -0.9999939076577903929, -0.003490651415223739937 ) ) ;
#107962=ADVANCED_FACE ( 'NONE', ( #65120 ), #33879, .T. ) ;
#107963=AXIS2_PLACEMENT_3D ( 'NONE', #108160, #127809, #37514 ) ;
#107964=ORIENTED_EDGE ( 'NONE', *, *, #13520, .T. ) ;
#107965=CARTESIAN_POINT ( 'NONE',  ( 1.449999999999952216, 12.50000000000000000, -2.576566944158915184 ) ) ;
#107966=CARTESIAN_POINT ( 'NONE',  ( 17.50000000000000000, -0.9166666666666694052, -3.999999999999998224 ) ) ;
#107969=DIRECTION ( 'NONE',  ( 0.000000000000000000, 1.000000000000000000, 0.000000000000000000 ) ) ;
#107970=ORIENTED_EDGE ( 'NONE', *, *, #49592, .T. ) ;
#107971=LINE ( 'NONE', #18292, #30645 ) ;
#107972=DIRECTION ( 'NONE',  ( -0.000000000000000000, -1.000000000000000000, -0.000000000000000000 ) ) ;
#107973=ORIENTED_EDGE ( 'NONE', *, *, #22890, .F. ) ;
#107974=EDGE_LOOP ( 'NONE', ( #121650, #52926, #115615, #15261 ) ) ;
#107975=ORIENTED_EDGE ( 'NONE', *, *, #72991, .F. ) ;
#107976=DIRECTION ( 'NONE',  ( -0.000000000000000000, -1.000000000000000000, -0.000000000000000000 ) ) ;
#107977=DIRECTION ( 'NONE',  ( -0.000000000000000000, -1.000000000000000000, -0.000000000000000000 ) ) ;
#107979=CARTESIAN_POINT ( 'NONE',  ( 12.29999999999990301, 2.500000000000000000, -0.4464101615137782142 ) ) ;
#107980=DIRECTION ( 'NONE',  ( 0.000000000000000000, 0.000000000000000000, 1.000000000000000000 ) ) ;
#107981=DIRECTION ( 'NONE',  ( 0.000000000000000000, 0.000000000000000000, 1.000000000000000000 ) ) ;
#107982=DIRECTION ( 'NONE',  ( 0.000000000000000000, -0.9999939076577903929, 0.003490651415223739937 ) ) ;
#107983=EDGE_LOOP ( 'NONE', ( #30378, #51915 ) ) ;
#107984=DIRECTION ( 'NONE',  ( 0.000000000000000000, 0.000000000000000000, -1.000000000000000000 ) ) ;
#107985=EDGE_CURVE ( 'NONE', #17292, #124192, #73577, .T. ) ;
#107986=VECTOR ( 'NONE', #34081, 1000.000000000000000 ) ;
#107987=ORIENTED_EDGE ( 'NONE', *, *, #89318, .T. ) ;
#107988=ORIENTED_EDGE ( 'NONE', *, *, #38696, .F. ) ;
#107989=CARTESIAN_POINT ( 'NONE',  ( 9.599999999999914380, 12.50000000000000000, -4.330127018922201643 ) ) ;
#107990=CARTESIAN_POINT ( 'NONE',  ( -2.300000000000033573, 2.500000000000000000, 0.2464101615137735679 ) ) ;
#107991=FACE_BOUND ( 'NONE', #127101, .T. ) ;
#107992=DIRECTION ( 'NONE',  ( 0.000000000000000000, 1.000000000000000000, 0.000000000000000000 ) ) ;
#107993=CARTESIAN_POINT ( 'NONE',  ( 14.39999999999989555, 2.500000000000000000, -0.3464101615137782364 ) ) ;
#107994=AXIS2_PLACEMENT_3D ( 'NONE', #2675, #94286, #55008 ) ;
#107996=FACE_OUTER_BOUND ( 'NONE', #96130, .T. ) ;
#107997=EDGE_CURVE ( 'NONE', #24704, #109720, #95893, .T. ) ;
#107998=ORIENTED_EDGE ( 'NONE', *, *, #10116, .T. ) ;
#108000=FACE_OUTER_BOUND ( 'NONE', #16968, .T. ) ;
#108001=FACE_OUTER_BOUND ( 'NONE', #22392, .T. ) ;
#108002=DIRECTION ( 'NONE',  ( 0.000000000000000000, 0.000000000000000000, 1.000000000000000000 ) ) ;
#108003=ORIENTED_EDGE ( 'NONE', *, *, #544, .T. ) ;
#108004=AXIS2_PLACEMENT_3D ( 'NONE', #117160, #58281, #118469 ) ;
#108005=CARTESIAN_POINT ( 'NONE',  ( -3.642919299551294898E-14, 12.50000000000000000, 0.7579135962115892688 ) ) ;
#108006=VECTOR ( 'NONE', #26785, 1000.000000000000000 ) ;
#108007=DIRECTION ( 'NONE',  ( -0.000000000000000000, -1.000000000000000000, -0.000000000000000000 ) ) ;
#108008=ORIENTED_EDGE ( 'NONE', *, *, #127276, .T. ) ;
#108009=ORIENTED_EDGE ( 'NONE', *, *, #107902, .T. ) ;
#108010=DIRECTION ( 'NONE',  ( -0.000000000000000000, -1.000000000000000000, -0.000000000000000000 ) ) ;
#108011=FACE_OUTER_BOUND ( 'NONE', #29006, .T. ) ;
#108012=FACE_BOUND ( 'NONE', #44465, .T. ) ;
#108013=FACE_OUTER_BOUND ( 'NONE', #78228, .T. ) ;
#108014=ORIENTED_EDGE ( 'NONE', *, *, #76917, .F. ) ;
#108015=FACE_OUTER_BOUND ( 'NONE', #48932, .T. ) ;
#108016=ORIENTED_EDGE ( 'NONE', *, *, #93006, .T. ) ;
#108017=EDGE_LOOP ( 'NONE', ( #108364, #30610, #46275, #46061 ) ) ;
#108018=DIRECTION ( 'NONE',  ( -0.000000000000000000, -1.000000000000000000, -0.000000000000000000 ) ) ;
#108020=AXIS2_PLACEMENT_3D ( 'NONE', #88064, #39671, #128024 ) ;
#108021=VECTOR ( 'NONE', #5972, 1000.000000000000000 ) ;
#108022=VERTEX_POINT ( 'NONE', #105719 ) ;
#108023=CARTESIAN_POINT ( 'NONE',  ( 3.099999999999943245, 2.500000000000000000, 4.083716857408420609 ) ) ;
#108024=VECTOR ( 'NONE', #97744, 1000.000000000000000 ) ;
#108025=LINE ( 'NONE', #78596, #23976 ) ;
#108026=EDGE_CURVE ( 'NONE', #92529, #76531, #50603, .T. ) ;
#108027=FACE_OUTER_BOUND ( 'NONE', #91645, .T. ) ;
#108028=DIRECTION ( 'NONE',  ( 0.000000000000000000, -0.9999939076577903929, 0.003490651415223739937 ) ) ;
#108029=AXIS2_PLACEMENT_3D ( 'NONE', #122215, #32561, #72469 ) ;
#108030=AXIS2_PLACEMENT_3D ( 'NONE', #113995, #117022, #117662 ) ;
#108031=EDGE_CURVE ( 'NONE', #37336, #6486, #35691, .T. ) ;
#108032=ORIENTED_EDGE ( 'NONE', *, *, #116238, .T. ) ;
#108033=DIRECTION ( 'NONE',  ( 0.000000000000000000, 0.000000000000000000, 1.000000000000000000 ) ) ;
#108034=CARTESIAN_POINT ( 'NONE',  ( 13.09999999999989839, 2.500000000000000000, -0.3464101615137783474 ) ) ;
#108035=ORIENTED_EDGE ( 'NONE', *, *, #55764, .T. ) ;
#108036=EDGE_CURVE ( 'NONE', #116926, #107710, #123744, .T. ) ;
#108037=DIRECTION ( 'NONE',  ( 0.000000000000000000, 0.000000000000000000, 1.000000000000000000 ) ) ;
#108038=ORIENTED_EDGE ( 'NONE', *, *, #35271, .F. ) ;
#108039=AXIS2_PLACEMENT_3D ( 'NONE', #19023, #81816, #52366 ) ;
#108040=ADVANCED_FACE ( 'NONE', ( #27149 ), #56589, .T. ) ;
#108041=PLANE ( 'NONE',  #88984 ) ;
#108042=CONICAL_SURFACE ( 'NONE', #39129, 0.1000000000000002554, 0.003490658503988666988 ) ;
#108043=VERTEX_POINT ( 'NONE', #18615 ) ;
#108044=FACE_OUTER_BOUND ( 'NONE', #94800, .T. ) ;
#108046=LINE ( 'NONE', #61380, #35069 ) ;
#108047=AXIS2_PLACEMENT_3D ( 'NONE', #89411, #39695, #10207 ) ;
#108048=VECTOR ( 'NONE', #13856, 1000.000000000000000 ) ;
#108049=DIRECTION ( 'NONE',  ( 0.000000000000000000, 1.000000000000000000, 0.000000000000000000 ) ) ;
#108050=ORIENTED_EDGE ( 'NONE', *, *, #48861, .T. ) ;
#108051=ADVANCED_FACE ( 'NONE', ( #96507 ), #100860, .T. ) ;
#108052=CARTESIAN_POINT ( 'NONE',  ( 0.8499999999999553468, 2.500000000000000000, -2.957883832488653830 ) ) ;
#108053=DIRECTION ( 'NONE',  ( 0.000000000000000000, -0.000000000000000000, 1.000000000000000000 ) ) ;
#108054=DIRECTION ( 'NONE',  ( 0.000000000000000000, -0.9999939076577903929, 0.003490651415223739937 ) ) ;
#108055=DIRECTION ( 'NONE',  ( 0.000000000000000000, 0.000000000000000000, -1.000000000000000000 ) ) ;
#108056=CARTESIAN_POINT ( 'NONE',  ( -6.083778633910298187E-15, 2.500000000000000000, -4.430127018922202176 ) ) ;
#108057=EDGE_CURVE ( 'NONE', #82164, #13480, #57260, .T. ) ;
#108058=DIRECTION ( 'NONE',  ( -0.000000000000000000, -1.000000000000000000, -0.000000000000000000 ) ) ;
#108059=EDGE_LOOP ( 'NONE', ( #104629, #89230, #75259, #16077 ) ) ;
#108060=ORIENTED_EDGE ( 'NONE', *, *, #90340, .F. ) ;
#108061=CARTESIAN_POINT ( 'NONE',  ( -9.400000000000007461, 2.500000000000000000, 0.3464101615137735735 ) ) ;
#108062=ORIENTED_EDGE ( 'NONE', *, *, #84585, .F. ) ;
#108063=FACE_OUTER_BOUND ( 'NONE', #12170, .T. ) ;
#108064=ORIENTED_EDGE ( 'NONE', *, *, #77187, .T. ) ;
#108065=ORIENTED_EDGE ( 'NONE', *, *, #7231, .F. ) ;
#108066=VERTEX_POINT ( 'NONE', #6833 ) ;
#108067=CIRCLE ( 'NONE', #51652, 0.1000000000000000472 ) ;
#108068=CARTESIAN_POINT ( 'NONE',  ( 17.50000000000000000, 2.500000000000000000, -3.999999999999996447 ) ) ;
#108069=CARTESIAN_POINT ( 'NONE',  ( 6.849999999999929479, 12.50000000000000000, 6.841600689897072485 ) ) ;
#108070=DIRECTION ( 'NONE',  ( 0.000000000000000000, 0.000000000000000000, 1.000000000000000000 ) ) ;
#108072=DIRECTION ( 'NONE',  ( 0.000000000000000000, -0.000000000000000000, 1.000000000000000000 ) ) ;
#108073=CARTESIAN_POINT ( 'NONE',  ( -0.4000000000000331624, 12.50000000000000000, -0.6928203230275519209 ) ) ;
#108074=DIRECTION ( 'NONE',  ( 0.000000000000000000, 1.000000000000000000, 0.000000000000000000 ) ) ;
#108075=ORIENTED_EDGE ( 'NONE', *, *, #43107, .T. ) ;
#108076=ORIENTED_EDGE ( 'NONE', *, *, #100518, .F. ) ;
#108078=AXIS2_PLACEMENT_3D ( 'NONE', #67053, #83670, #33918 ) ;
#108079=FACE_OUTER_BOUND ( 'NONE', #96733, .T. ) ;
#108080=EDGE_LOOP ( 'NONE', ( #99339, #62607, #111496, #122584 ) ) ;
#108081=VERTEX_POINT ( 'NONE', #46801 ) ;
#108082=CONICAL_SURFACE ( 'NONE', #101838, 0.1000000000000000472, 0.003490658503988666988 ) ;
#108083=CIRCLE ( 'NONE', #101840, 0.1000000000000000056 ) ;
#108084=EDGE_CURVE ( 'NONE', #25178, #121192, #115518, .T. ) ;
#108085=DIRECTION ( 'NONE',  ( 0.000000000000000000, 0.000000000000000000, 1.000000000000000000 ) ) ;
#108086=CARTESIAN_POINT ( 'NONE',  ( -5.650000000000019895, 2.500000000000000000, 2.411473670974873862 ) ) ;
#108087=CARTESIAN_POINT ( 'NONE',  ( 10.84999999999991260, 2.500000000000000000, 6.395190528383296602 ) ) ;
#108088=FACE_OUTER_BOUND ( 'NONE', #112187, .T. ) ;
#108089=EDGE_CURVE ( 'NONE', #5141, #22283, #46482, .T. ) ;
#108090=CARTESIAN_POINT ( 'NONE',  ( -11.05000000000000071, 2.500000000000000000, 6.941600689897073018 ) ) ;
#108091=ORIENTED_EDGE ( 'NONE', *, *, #6121, .T. ) ;
#108092=EDGE_CURVE ( 'NONE', #76885, #45239, #30247, .T. ) ;
#108093=ADVANCED_FACE ( 'NONE', ( #76896 ), #84132, .T. ) ;
#108095=AXIS2_PLACEMENT_3D ( 'NONE', #25521, #127451, #8940 ) ;
#108096=AXIS2_PLACEMENT_3D ( 'NONE', #67928, #47020, #77732 ) ;
#108097=EDGE_CURVE ( 'NONE', #37483, #129577, #16658, .T. ) ;
#108098=ORIENTED_EDGE ( 'NONE', *, *, #82421, .T. ) ;
#108099=DIRECTION ( 'NONE',  ( 0.000000000000000000, 0.000000000000000000, 1.000000000000000000 ) ) ;
#108101=ORIENTED_EDGE ( 'NONE', *, *, #89155, .T. ) ;
#108102=CARTESIAN_POINT ( 'NONE',  ( 4.799999999999935874, 2.500000000000000000, 0.3464101615137735735 ) ) ;
#108103=EDGE_CURVE ( 'NONE', #127931, #78711, #23501, .T. ) ;
#108104=VERTEX_POINT ( 'NONE', #37628 ) ;
#108105=ORIENTED_EDGE ( 'NONE', *, *, #46582, .F. ) ;
#108106=LINE ( 'NONE', #116635, #98417 ) ;
#108107=CARTESIAN_POINT ( 'NONE',  ( -11.89999999999999680, 2.500000000000000000, -3.983716857408423628 ) ) ;
#108108=EDGE_CURVE ( 'NONE', #7764, #33696, #27702, .T. ) ;
#108109=EDGE_CURVE ( 'NONE', #124470, #60953, #102925, .T. ) ;
#108110=CARTESIAN_POINT ( 'NONE',  ( -9.200000000000009948, 12.50000000000000000, -4.395220292106235327 ) ) ;
#108111=LINE ( 'NONE', #127757, #126234 ) ;
#108112=DIRECTION ( 'NONE',  ( 0.000000000000000000, 0.000000000000000000, 1.000000000000000000 ) ) ;
#108113=VERTEX_POINT ( 'NONE', #19920 ) ;
#108114=CARTESIAN_POINT ( 'NONE',  ( -5.200000000000024158, 2.500000000000000000, -4.776537180435977525 ) ) ;
#108115=DIRECTION ( 'NONE',  ( 0.000000000000000000, 0.000000000000000000, 1.000000000000000000 ) ) ;
#108116=FACE_OUTER_BOUND ( 'NONE', #61843, .T. ) ;
#108117=DIRECTION ( 'NONE',  ( -0.000000000000000000, -1.000000000000000000, -0.000000000000000000 ) ) ;
#108118=CIRCLE ( 'NONE', #83009, 0.06509327318403745899 ) ;
#108119=CONICAL_SURFACE ( 'NONE', #20300, 0.1000000000000000472, 0.003490658503988666988 ) ;
#108120=CARTESIAN_POINT ( 'NONE',  ( 8.149999999999920419, 12.50000000000000000, -1.818653347947325916 ) ) ;
#108121=ORIENTED_EDGE ( 'NONE', *, *, #66578, .F. ) ;
#108122=AXIS2_PLACEMENT_3D ( 'NONE', #104303, #15906, #95768 ) ;
#108123=VERTEX_POINT ( 'NONE', #50041 ) ;
#108124=DIRECTION ( 'NONE',  ( 0.000000000000000000, -0.9999939076577903929, 0.003490651415223739937 ) ) ;
#108125=ADVANCED_FACE ( 'NONE', ( #120689 ), #11373, .T. ) ;
#108126=CIRCLE ( 'NONE', #83102, 0.06509327318403741736 ) ;
#108127=ORIENTED_EDGE ( 'NONE', *, *, #2434, .F. ) ;
#108128=CONICAL_SURFACE ( 'NONE', #51706, 0.1000000000000002554, 0.003490658503988666988 ) ;
#108129=DIRECTION ( 'NONE',  ( 0.000000000000000000, 1.000000000000000000, 0.000000000000000000 ) ) ;
#108131=CIRCLE ( 'NONE', #110281, 0.1000000000000002554 ) ;
#108132=AXIS2_PLACEMENT_3D ( 'NONE', #68698, #36024, #107980 ) ;
#108133=VERTEX_POINT ( 'NONE', #70305 ) ;
#108135=CARTESIAN_POINT ( 'NONE',  ( -15.79999999999998117, 2.500000000000000000, 0.1000000000000000056 ) ) ;
#108136=PLANE ( 'NONE',  #52432 ) ;
#108137=DIRECTION ( 'NONE',  ( 0.000000000000000000, 0.000000000000000000, 1.000000000000000000 ) ) ;
#108138=VERTEX_POINT ( 'NONE', #19242 ) ;
#108139=CIRCLE ( 'NONE', #110210, 0.06509327318403745899 ) ;
#108140=AXIS2_PLACEMENT_3D ( 'NONE', #37387, #7246, #21433 ) ;
#108141=DIRECTION ( 'NONE',  ( 0.000000000000000000, 0.000000000000000000, -1.000000000000000000 ) ) ;
#108142=VERTEX_POINT ( 'NONE', #68999 ) ;
#108143=FACE_OUTER_BOUND ( 'NONE', #93679, .T. ) ;
#108144=CARTESIAN_POINT ( 'NONE',  ( 0.1999999999999567124, 2.500000000000000000, -3.883716857408426648 ) ) ;
#108145=CARTESIAN_POINT ( 'NONE',  ( 3.949999999999942446, 2.500000000000000000, -6.841600689897078702 ) ) ;
#108146=ADVANCED_FACE ( 'NONE', ( #1548 ), #128071, .T. ) ;
#108147=ORIENTED_EDGE ( 'NONE', *, *, #100125, .F. ) ;
#108148=DIRECTION ( 'NONE',  ( -4.274815082592931898E-19, -0.9999939076577903929, -0.003490651415223739937 ) ) ;
#108149=ORIENTED_EDGE ( 'NONE', *, *, #111527, .F. ) ;
#108150=CARTESIAN_POINT ( 'NONE',  ( 5.849999999999935696, 2.500000000000000000, -7.288010851410854585 ) ) ;
#108151=DIRECTION ( 'NONE',  ( -4.274815082592931898E-19, -0.9999939076577903929, -0.003490651415223739937 ) ) ;
#108152=AXIS2_PLACEMENT_3D ( 'NONE', #106233, #125856, #18486 ) ;
#108153=CARTESIAN_POINT ( 'NONE',  ( -14.14999999999998792, 2.500000000000000000, 2.757883832488653209 ) ) ;
#108154=ORIENTED_EDGE ( 'NONE', *, *, #18822, .F. ) ;
#108155=PLANE ( 'NONE',  #80242 ) ;
#108156=LINE ( 'NONE', #7374, #24507 ) ;
#108157=EDGE_LOOP ( 'NONE', ( #29485, #83402 ) ) ;
#108158=CARTESIAN_POINT ( 'NONE',  ( 8.099999999999923261, 12.50000000000000000, -4.611443907251940644 ) ) ;
#108159=ORIENTED_EDGE ( 'NONE', *, *, #38536, .T. ) ;
#108160=CARTESIAN_POINT ( 'NONE',  ( 8.149999999999920419, 2.500000000000000000, 6.841600689897072485 ) ) ;
#108161=CONICAL_SURFACE ( 'NONE', #72678, 0.1000000000000000056, 0.003490658503988666988 ) ;
#108162=VECTOR ( 'NONE', #125208, 1000.000000000000000 ) ;
#108163=ORIENTED_EDGE ( 'NONE', *, *, #60418, .F. ) ;
#108164=CARTESIAN_POINT ( 'NONE',  ( 9.999999999999911182, 12.50000000000000000, 5.022947341949748790 ) ) ;
#108165=FACE_OUTER_BOUND ( 'NONE', #63796, .T. ) ;
#108166=VERTEX_POINT ( 'NONE', #252 ) ;
#108167=ORIENTED_EDGE ( 'NONE', *, *, #121793, .T. ) ;
#108168=DIRECTION ( 'NONE',  ( 0.000000000000000000, 0.000000000000000000, 1.000000000000000000 ) ) ;
#108169=CARTESIAN_POINT ( 'NONE',  ( -3.950000000000026379, 12.50000000000000000, 2.511473670974873507 ) ) ;
#108170=ORIENTED_EDGE ( 'NONE', *, *, #109584, .F. ) ;
#108171=CIRCLE ( 'NONE', #20364, 0.09999999999999982514 ) ;
#108174=AXIS2_PLACEMENT_3D ( 'NONE', #44657, #6618, #104211 ) ;
#108176=CARTESIAN_POINT ( 'NONE',  ( -8.100000000000013856, 2.500000000000000000, -3.883716857408426648 ) ) ;
#108177=DIRECTION ( 'NONE',  ( -4.274815082592931898E-19, -0.9999939076577903929, -0.003490651415223739937 ) ) ;
#108178=DIRECTION ( 'NONE',  ( 0.000000000000000000, 0.000000000000000000, -1.000000000000000000 ) ) ;
#108179=CIRCLE ( 'NONE', #7546, 0.1000000000000000056 ) ;
#108180=CIRCLE ( 'NONE', #47570, 0.1000000000000002554 ) ;
#108181=EDGE_CURVE ( 'NONE', #65792, #86833, #96646, .T. ) ;
#108182=EDGE_LOOP ( 'NONE', ( #97236, #61100 ) ) ;
#108183=ORIENTED_EDGE ( 'NONE', *, *, #128649, .F. ) ;
#108184=VERTEX_POINT ( 'NONE', #10702 ) ;
#108185=VERTEX_POINT ( 'NONE', #80779 ) ;
#108186=DIRECTION ( 'NONE',  ( 0.000000000000000000, 0.000000000000000000, -1.000000000000000000 ) ) ;
#108187=DIRECTION ( 'NONE',  ( -4.274815082592931898E-19, -0.9999939076577903929, -0.003490651415223739937 ) ) ;
#108188=DIRECTION ( 'NONE',  ( 0.000000000000000000, 0.000000000000000000, 1.000000000000000000 ) ) ;
#108190=EDGE_CURVE ( 'NONE', #56111, #40454, #89292, .T. ) ;
#108191=FACE_BOUND ( 'NONE', #48931, .T. ) ;
#108192=EDGE_LOOP ( 'NONE', ( #22861, #4083 ) ) ;
#108193=ADVANCED_FACE ( 'NONE', ( #41509 ), #67381, .T. ) ;
#108194=DIRECTION ( 'NONE',  ( -0.000000000000000000, -1.000000000000000000, -0.000000000000000000 ) ) ;
#108195=CARTESIAN_POINT ( 'NONE',  ( -8.750000000000010658, 12.50000000000000000, 2.857883832488649301 ) ) ;
#108196=DIRECTION ( 'NONE',  ( 0.000000000000000000, 0.000000000000000000, 1.000000000000000000 ) ) ;
#108197=CIRCLE ( 'NONE', #83088, 0.1000000000000002554 ) ;
#108198=DIRECTION ( 'NONE',  ( 0.000000000000000000, 1.000000000000000000, 0.000000000000000000 ) ) ;
#108199=DIRECTION ( 'NONE',  ( -0.000000000000000000, -1.000000000000000000, -0.000000000000000000 ) ) ;
#108200=CONICAL_SURFACE ( 'NONE', #28799, 0.1000000000000000472, 0.003490658503988666988 ) ;
#108201=EDGE_CURVE ( 'NONE', #51148, #121928, #50655, .T. ) ;
#108202=CARTESIAN_POINT ( 'NONE',  ( -6.700000000000016165, 2.500000000000000000, 4.230127018922196669 ) ) ;
#108203=EDGE_CURVE ( 'NONE', #22700, #52514, #117566, .T. ) ;
#108204=DIRECTION ( 'NONE',  ( -0.000000000000000000, -1.000000000000000000, -0.000000000000000000 ) ) ;
#108205=CARTESIAN_POINT ( 'NONE',  ( 14.99999999999989342, 2.500000000000000000, -0.5928203230275541635 ) ) ;
#108206=ADVANCED_FACE ( 'NONE', ( #70941 ), #78852, .T. ) ;
#108207=DIRECTION ( 'NONE',  ( 0.000000000000000000, 0.000000000000000000, -1.000000000000000000 ) ) ;
#108208=ADVANCED_FACE ( 'NONE', ( #31664 ), #21192, .T. ) ;
#108209=AXIS2_PLACEMENT_3D ( 'NONE', #55275, #95196, #70546 ) ;
#108210=VECTOR ( 'NONE', #51091, 1000.000000000000000 ) ;
#108211=CARTESIAN_POINT ( 'NONE',  ( -2.500000000000032419, 2.500000000000000000, 0.7928203230275495672 ) ) ;
#108212=ORIENTED_EDGE ( 'NONE', *, *, #31810, .F. ) ;
#108213=CIRCLE ( 'NONE', #14109, 0.1000000000000000472 ) ;
#108214=ORIENTED_EDGE ( 'NONE', *, *, #73862, .F. ) ;
#108215=EDGE_LOOP ( 'NONE', ( #7257, #16357 ) ) ;
#108216=ORIENTED_EDGE ( 'NONE', *, *, #72482, .F. ) ;
#108217=CARTESIAN_POINT ( 'NONE',  ( 17.50011901588668906, -2.224285231025419307, -4.071013062218297840 ) ) ;
#108218=DIRECTION ( 'NONE',  ( -0.000000000000000000, 1.000000000000000000, -0.000000000000000000 ) ) ;
#108219=ORIENTED_EDGE ( 'NONE', *, *, #115899, .T. ) ;
#108220=EDGE_LOOP ( 'NONE', ( #103212, #24168, #104660, #101720 ) ) ;
#108221=EDGE_CURVE ( 'NONE', #120555, #37733, #29765, .T. ) ;
#108222=VECTOR ( 'NONE', #80042, 1000.000000000000000 ) ;
#108223=ORIENTED_EDGE ( 'NONE', *, *, #83031, .T. ) ;
#108224=DIRECTION ( 'NONE',  ( 0.000000000000000000, 1.000000000000000000, 0.000000000000000000 ) ) ;
#108225=AXIS2_PLACEMENT_3D ( 'NONE', #78282, #90657, #8222 ) ;
#108226=AXIS2_PLACEMENT_3D ( 'NONE', #66611, #67901, #96074 ) ;
#108227=DIRECTION ( 'NONE',  ( 0.000000000000000000, -0.000000000000000000, 1.000000000000000000 ) ) ;
#108229=FACE_OUTER_BOUND ( 'NONE', #80656, .T. ) ;
#108230=DIRECTION ( 'NONE',  ( 0.000000000000000000, -0.9999939076577903929, 0.003490651415223739937 ) ) ;
#108231=DIRECTION ( 'NONE',  ( 0.000000000000000000, 0.000000000000000000, 1.000000000000000000 ) ) ;
#108232=DIRECTION ( 'NONE',  ( 0.000000000000000000, 1.000000000000000000, 0.000000000000000000 ) ) ;
#108233=AXIS2_PLACEMENT_3D ( 'NONE', #127403, #126764, #37735 ) ;
#108234=VERTEX_POINT ( 'NONE', #69650 ) ;
#108235=DIRECTION ( 'NONE',  ( 0.000000000000000000, 1.000000000000000000, 0.000000000000000000 ) ) ;
#108236=VERTEX_POINT ( 'NONE', #118747 ) ;
#108237=CIRCLE ( 'NONE', #68519, 0.09999999999999982514 ) ;
#108238=CONICAL_SURFACE ( 'NONE', #122920, 0.1000000000000000056, 0.003490658503988666988 ) ;
#108239=VERTEX_POINT ( 'NONE', #71582 ) ;
#108240=ORIENTED_EDGE ( 'NONE', *, *, #41875, .F. ) ;
#108241=LINE ( 'NONE', #68962, #98483 ) ;
#108242=ORIENTED_EDGE ( 'NONE', *, *, #16732, .T. ) ;
#108243=ORIENTED_EDGE ( 'NONE', *, *, #91001, .F. ) ;
#108244=CARTESIAN_POINT ( 'NONE',  ( 2.299999999999947864, 12.50000000000000000, 4.048810130592458201 ) ) ;
#108245=CARTESIAN_POINT ( 'NONE',  ( 5.849999999999933920, 2.500000000000000000, -2.857883832488653741 ) ) ;
#108246=DIRECTION ( 'NONE',  ( 0.000000000000000000, 1.000000000000000000, 0.000000000000000000 ) ) ;
#108247=DIRECTION ( 'NONE',  ( -0.000000000000000000, -1.000000000000000000, -0.000000000000000000 ) ) ;
#108248=CARTESIAN_POINT ( 'NONE',  ( -8.950000000000009948, 2.500000000000000000, 2.511473670974873507 ) ) ;
#108249=ADVANCED_FACE ( 'NONE', ( #89927 ), #19286, .T. ) ;
#108250=ORIENTED_EDGE ( 'NONE', *, *, #25982, .T. ) ;
#108251=EDGE_CURVE ( 'NONE', #122621, #13831, #109170, .T. ) ;
#108252=CARTESIAN_POINT ( 'NONE',  ( -10.85000000000000142, 2.500000000000000000, -6.495190528383298911 ) ) ;
#108253=EDGE_LOOP ( 'NONE', ( #87764, #23984, #77855, #59515 ) ) ;
#108254=CARTESIAN_POINT ( 'NONE',  ( 16.56034314470449686, 0.8287381876616523035, 6.090234461610898542 ) ) ;
#108255=EDGE_CURVE ( 'NONE', #125293, #61342, #54894, .T. ) ;
#108256=ORIENTED_EDGE ( 'NONE', *, *, #68032, .T. ) ;
#108258=DIRECTION ( 'NONE',  ( 0.000000000000000000, 0.000000000000000000, -1.000000000000000000 ) ) ;
#108259=ORIENTED_EDGE ( 'NONE', *, *, #119262, .T. ) ;
#108260=LINE ( 'NONE', #78828, #71833 ) ;
#108261=AXIS2_PLACEMENT_3D ( 'NONE', #43042, #100625, #2416 ) ;
#108262=EDGE_CURVE ( 'NONE', #45293, #24007, #88649, .T. ) ;
#108263=FACE_OUTER_BOUND ( 'NONE', #86277, .T. ) ;
#108264=EDGE_LOOP ( 'NONE', ( #109394, #105336, #22720, #49685 ) ) ;
#108265=ADVANCED_FACE ( 'NONE', ( #40200 ), #93175, .T. ) ;
#108266=AXIS2_PLACEMENT_3D ( 'NONE', #37427, #28241, #68803 ) ;
#108268=CIRCLE ( 'NONE', #51842, 0.1000000000000002554 ) ;
#108269=ADVANCED_FACE ( 'NONE', ( #94434 ), #94596, .T. ) ;
#108270=CARTESIAN_POINT ( 'NONE',  ( 4.149999999999939959, 2.500000000000000000, -6.395190528383301931 ) ) ;
#108271=EDGE_LOOP ( 'NONE', ( #117141, #77168 ) ) ;
#108272=ORIENTED_EDGE ( 'NONE', *, *, #68196, .F. ) ;
#108273=CARTESIAN_POINT ( 'NONE',  ( 11.44999999999990870, 2.500000000000000000, -1.818653347947326138 ) ) ;
#108274=CARTESIAN_POINT ( 'NONE',  ( -13.14999999999999147, 12.50000000000000000, -1.818653347947323917 ) ) ;
#108276=PLANE ( 'NONE',  #126505 ) ;
#108277=ADVANCED_FACE ( 'NONE', ( #113440 ), #64342, .T. ) ;
#108278=VECTOR ( 'NONE', #33419, 1000.000000000000000 ) ;
#108279=DIRECTION ( 'NONE',  ( -4.274815082592931898E-19, -0.9999939076577903929, -0.003490651415223739937 ) ) ;
#108280=CIRCLE ( 'NONE', #76979, 0.1000000000000002554 ) ;
#108281=ORIENTED_EDGE ( 'NONE', *, *, #86781, .T. ) ;
#108282=DIRECTION ( 'NONE',  ( -0.000000000000000000, 1.000000000000000000, -0.000000000000000000 ) ) ;
#108283=CARTESIAN_POINT ( 'NONE',  ( 4.149999999999936406, 2.500000000000000000, 6.595190528383296780 ) ) ;
#108284=AXIS2_PLACEMENT_3D ( 'NONE', #107394, #126396, #77931 ) ;
#108285=EDGE_LOOP ( 'NONE', ( #25208, #119738 ) ) ;
#108286=AXIS2_PLACEMENT_3D ( 'NONE', #17285, #87329, #109570 ) ;
#108287=FACE_OUTER_BOUND ( 'NONE', #20712, .T. ) ;
#108288=FACE_OUTER_BOUND ( 'NONE', #110137, .T. ) ;
#108289=DIRECTION ( 'NONE',  ( 0.000000000000000000, -0.000000000000000000, 1.000000000000000000 ) ) ;
#108291=PLANE ( 'NONE',  #51668 ) ;
#108292=ORIENTED_EDGE ( 'NONE', *, *, #89684, .T. ) ;
#108293=AXIS2_PLACEMENT_3D ( 'NONE', #90119, #77724, #29301 ) ;
#108294=CARTESIAN_POINT ( 'NONE',  ( 1.649999999999951505, 12.50000000000000000, 2.857883832488649301 ) ) ;
#108295=DIRECTION ( 'NONE',  ( 0.000000000000000000, -0.9999939076577903929, 0.003490651415223739937 ) ) ;
#108296=AXIS2_PLACEMENT_3D ( 'NONE', #10644, #90516, #80718 ) ;
#108297=AXIS2_PLACEMENT_3D ( 'NONE', #11324, #40810, #68953 ) ;
#108298=VERTEX_POINT ( 'NONE', #14579 ) ;
#108299=LINE ( 'NONE', #86729, #94892 ) ;
#108300=AXIS2_PLACEMENT_3D ( 'NONE', #68213, #57769, #38122 ) ;
#108301=ADVANCED_FACE ( 'NONE', ( #43439 ), #119640, .T. ) ;
#108302=EDGE_LOOP ( 'NONE', ( #111771, #119314, #21292, #43536 ) ) ;
#108303=ORIENTED_EDGE ( 'NONE', *, *, #121527, .T. ) ;
#108304=DIRECTION ( 'NONE',  ( 0.000000000000000000, 0.000000000000000000, 1.000000000000000000 ) ) ;
#108305=CONICAL_SURFACE ( 'NONE', #95793, 0.1000000000000000472, 0.003490658503988666988 ) ;
#108306=ORIENTED_EDGE ( 'NONE', *, *, #28324, .F. ) ;
#108307=PLANE ( 'NONE',  #125973 ) ;
#108308=PLANE ( 'NONE',  #102823 ) ;
#108309=CARTESIAN_POINT ( 'NONE',  ( 4.399999999999940847, 2.500000000000000000, -3.983716857408426293 ) ) ;
#108310=ORIENTED_EDGE ( 'NONE', *, *, #109888, .T. ) ;
#108311=CARTESIAN_POINT ( 'NONE',  ( -11.89999999999999680, 2.500000000000000000, -4.676537180435976104 ) ) ;
#108312=DIRECTION ( 'NONE',  ( 0.000000000000000000, -0.9999939076577903929, 0.003490651415223739937 ) ) ;
#108313=EDGE_LOOP ( 'NONE', ( #6488, #13697, #3515, #19024 ) ) ;
#108314=CARTESIAN_POINT ( 'NONE',  ( 12.09999999999990550, 12.50000000000000000, -5.022947341949754119 ) ) ;
#108315=CIRCLE ( 'NONE', #129280, 0.1000000000000002554 ) ;
#108316=ADVANCED_FACE ( 'NONE', ( #63708 ), #3491, .T. ) ;
#108317=PLANE ( 'NONE',  #124113 ) ;
#108318=ORIENTED_EDGE ( 'NONE', *, *, #75131, .F. ) ;
#108319=AXIS2_PLACEMENT_3D ( 'NONE', #61434, #68162, #108085 ) ;
#108320=AXIS2_PLACEMENT_3D ( 'NONE', #91087, #49894, #10573 ) ;
#108321=ORIENTED_EDGE ( 'NONE', *, *, #12659, .T. ) ;
#108322=ORIENTED_EDGE ( 'NONE', *, *, #10963, .F. ) ;
#108323=DIRECTION ( 'NONE',  ( -0.000000000000000000, 1.000000000000000000, -0.000000000000000000 ) ) ;
#108324=CARTESIAN_POINT ( 'NONE',  ( 10.39999999999991154, 2.500000000000000000, 5.022947341949748790 ) ) ;
#108325=DIRECTION ( 'NONE',  ( 0.000000000000000000, 1.000000000000000000, 0.000000000000000000 ) ) ;
#108326=FACE_BOUND ( 'NONE', #112763, .T. ) ;
#108327=EDGE_LOOP ( 'NONE', ( #43386, #51734 ) ) ;
#108328=DIRECTION ( 'NONE',  ( -0.000000000000000000, 1.000000000000000000, -0.000000000000000000 ) ) ;
#108329=DIRECTION ( 'NONE',  ( 0.000000000000000000, 0.000000000000000000, 1.000000000000000000 ) ) ;
#108330=VERTEX_POINT ( 'NONE', #92506 ) ;
#108332=DIRECTION ( 'NONE',  ( -4.274815082592931898E-19, -0.9999939076577903929, -0.003490651415223739937 ) ) ;
#108333=DIRECTION ( 'NONE',  ( -4.274815082592931898E-19, -0.9999939076577903929, -0.003490651415223739937 ) ) ;
#108334=DIRECTION ( 'NONE',  ( -0.000000000000000000, -1.000000000000000000, -0.000000000000000000 ) ) ;
#108335=CONICAL_SURFACE ( 'NONE', #10147, 0.1000000000000002554, 0.003490658503988666988 ) ;
#108336=CARTESIAN_POINT ( 'NONE',  ( -6.700000000000019718, 2.500000000000000000, -4.430127018922202176 ) ) ;
#108337=CARTESIAN_POINT ( 'NONE',  ( -5.200000000000024158, 12.50000000000000000, -4.676537180435977881 ) ) ;
#108338=DIRECTION ( 'NONE',  ( -4.274815082592931898E-19, -0.9999939076577903929, -0.003490651415223739937 ) ) ;
#108339=CIRCLE ( 'NONE', #70785, 0.1000000000000000472 ) ;
#108340=ADVANCED_FACE ( 'NONE', ( #22509 ), #102344, .T. ) ;
#108341=ORIENTED_EDGE ( 'NONE', *, *, #8610, .T. ) ;
#108342=ORIENTED_EDGE ( 'NONE', *, *, #51647, .F. ) ;
#108343=ORIENTED_EDGE ( 'NONE', *, *, #119114, .F. ) ;
#108344=CIRCLE ( 'NONE', #51934, 0.09999999999999982514 ) ;
#108345=EDGE_LOOP ( 'NONE', ( #206, #77796, #116321, #127521 ) ) ;
#108346=EDGE_LOOP ( 'NONE', ( #69632, #33488 ) ) ;
#108347=CARTESIAN_POINT ( 'NONE',  ( 8.349999999999923261, 2.500000000000000000, 2.857883832488649301 ) ) ;
#108348=DIRECTION ( 'NONE',  ( 0.000000000000000000, 0.000000000000000000, 1.000000000000000000 ) ) ;
#108349=EDGE_LOOP ( 'NONE', ( #104045, #95755, #113700, #4072 ) ) ;
#108350=FACE_BOUND ( 'NONE', #2871, .T. ) ;
#108351=EDGE_CURVE ( 'NONE', #80116, #118274, #79940, .T. ) ;
#108352=CARTESIAN_POINT ( 'NONE',  ( 5.399999999999936406, 2.500000000000000000, -3.737306695894649700 ) ) ;
#108353=AXIS2_PLACEMENT_3D ( 'NONE', #81508, #44645, #1638 ) ;
#108354=VECTOR ( 'NONE', #30187, 1000.000000000000000 ) ;
#108355=CONICAL_SURFACE ( 'NONE', #87420, 0.09999999999999982514, 0.003490658503988666988 ) ;
#108356=CARTESIAN_POINT ( 'NONE',  ( -0.8500000000000386136, 12.50000000000000000, 5.802370205355744659 ) ) ;
#108358=FACE_OUTER_BOUND ( 'NONE', #102991, .T. ) ;
#108359=EDGE_CURVE ( 'NONE', #40017, #71388, #124562, .T. ) ;
#108360=LINE ( 'NONE', #118183, #17778 ) ;
#108361=ADVANCED_FACE ( 'NONE', ( #121982 ), #13292, .T. ) ;
#108362=CARTESIAN_POINT ( 'NONE',  ( -5.400000000000019895, 12.50000000000000000, 3.572213422710607489 ) ) ;
#108363=EDGE_CURVE ( 'NONE', #62955, #112193, #56931, .T. ) ;
#108364=ORIENTED_EDGE ( 'NONE', *, *, #95842, .F. ) ;
#108365=ORIENTED_EDGE ( 'NONE', *, *, #42193, .F. ) ;
#108366=AXIS2_PLACEMENT_3D ( 'NONE', #10398, #90232, #88296 ) ;
#108367=VERTEX_POINT ( 'NONE', #62426 ) ;
#108368=ORIENTED_EDGE ( 'NONE', *, *, #117101, .T. ) ;
#108369=PLANE ( 'NONE',  #58944 ) ;
#108370=CARTESIAN_POINT ( 'NONE',  ( 13.91976764350745555, 2.499999999999999556, 6.779443706236890854 ) ) ;
#108371=CARTESIAN_POINT ( 'NONE',  ( -13.94999999999998863, 12.50000000000000000, 2.511473670974877503 ) ) ;
#108372=ORIENTED_EDGE ( 'NONE', *, *, #115908, .F. ) ;
#108373=EDGE_CURVE ( 'NONE', #104314, #43021, #54508, .T. ) ;
#108374=LINE ( 'NONE', #97905, #120761 ) ;
#108375=ADVANCED_FACE ( 'NONE', ( #114090 ), #101698, .T. ) ;
#108376=CIRCLE ( 'NONE', #28973, 0.06509327318403745899 ) ;
#108377=DIRECTION ( 'NONE',  ( 0.000000000000000000, 0.000000000000000000, 1.000000000000000000 ) ) ;
#108378=ADVANCED_FACE ( 'NONE', ( #23127 ), #80039, .T. ) ;
#108379=CARTESIAN_POINT ( 'NONE',  ( 8.349999999999923261, 12.50000000000000000, 2.165063509461097713 ) ) ;
#108381=DIRECTION ( 'NONE',  ( -0.000000000000000000, 1.000000000000000000, -0.000000000000000000 ) ) ;
#108382=CARTESIAN_POINT ( 'NONE',  ( -8.750000000000007105, 2.500000000000000000, 7.088010851410848190 ) ) ;
#108383=AXIS2_PLACEMENT_3D ( 'NONE', #75426, #93800, #106197 ) ;
#108384=CARTESIAN_POINT ( 'NONE',  ( -2.100000000000034728, 2.500000000000000000, 4.430127018922196847 ) ) ;
#108385=ORIENTED_EDGE ( 'NONE', *, *, #95642, .F. ) ;
#108386=DIRECTION ( 'NONE',  ( 0.000000000000000000, 0.000000000000000000, -1.000000000000000000 ) ) ;
#108387=VECTOR ( 'NONE', #124213, 1000.000000000000000 ) ;
#108388=VERTEX_POINT ( 'NONE', #47292 ) ;
#108389=VERTEX_POINT ( 'NONE', #78027 ) ;
#108390=DIRECTION ( 'NONE',  ( 0.000000000000000000, 0.000000000000000000, 1.000000000000000000 ) ) ;
#108391=DIRECTION ( 'NONE',  ( 0.000000000000000000, 0.000000000000000000, 1.000000000000000000 ) ) ;
#108392=DIRECTION ( 'NONE',  ( 0.000000000000000000, 0.000000000000000000, -1.000000000000000000 ) ) ;
#108393=ORIENTED_EDGE ( 'NONE', *, *, #50795, .T. ) ;
#108394=CONICAL_SURFACE ( 'NONE', #22741, 0.1000000000000002554, 0.003490658503988666988 ) ;
#108395=ORIENTED_EDGE ( 'NONE', *, *, #22714, .T. ) ;
#108396=DIRECTION ( 'NONE',  ( 0.000000000000000000, 0.000000000000000000, -1.000000000000000000 ) ) ;
#108397=CIRCLE ( 'NONE', #31063, 0.06509327318403745899 ) ;
#108398=DIRECTION ( 'NONE',  ( 0.000000000000000000, -0.000000000000000000, 1.000000000000000000 ) ) ;
#108399=CARTESIAN_POINT ( 'NONE',  ( -5.600000000000023626, 12.50000000000000000, -3.983716857408426293 ) ) ;
#108400=EDGE_LOOP ( 'NONE', ( #43373, #48407, #90549, #76727 ) ) ;
#108401=ORIENTED_EDGE ( 'NONE', *, *, #22219, .T. ) ;
#108402=DIRECTION ( 'NONE',  ( 0.000000000000000000, -0.000000000000000000, 1.000000000000000000 ) ) ;
#108403=ORIENTED_EDGE ( 'NONE', *, *, #129330, .F. ) ;
#108404=FACE_OUTER_BOUND ( 'NONE', #34277, .T. ) ;
#108405=ORIENTED_EDGE ( 'NONE', *, *, #37873, .T. ) ;
#108406=DIRECTION ( 'NONE',  ( -0.000000000000000000, -1.000000000000000000, -0.000000000000000000 ) ) ;
#108409=CONICAL_SURFACE ( 'NONE', #22759, 0.1000000000000002554, 0.003490658503988666988 ) ;
#108410=EDGE_CURVE ( 'NONE', #33730, #114232, #109276, .T. ) ;
#108411=DIRECTION ( 'NONE',  ( 0.000000000000000000, 0.000000000000000000, 1.000000000000000000 ) ) ;
#108412=ORIENTED_EDGE ( 'NONE', *, *, #104064, .T. ) ;
#108413=EDGE_CURVE ( 'NONE', #89818, #56893, #76744, .T. ) ;
#108414=CARTESIAN_POINT ( 'NONE',  ( 2.099999999999950351, 2.500000000000000000, -4.330127018922201643 ) ) ;
#108415=CIRCLE ( 'NONE', #104217, 0.06509327318403745899 ) ;
#108416=CIRCLE ( 'NONE', #51995, 0.09999999999999999167 ) ;
#108417=EDGE_CURVE ( 'NONE', #10886, #118566, #15876, .T. ) ;
#108418=ORIENTED_EDGE ( 'NONE', *, *, #108993, .F. ) ;
#108419=VERTEX_POINT ( 'NONE', #97024 ) ;
#108420=DIRECTION ( 'NONE',  ( 0.000000000000000000, 0.000000000000000000, 1.000000000000000000 ) ) ;
#108421=CARTESIAN_POINT ( 'NONE',  ( -10.40000000000000213, 12.50000000000000000, 4.395220292106234439 ) ) ;
#108422=DIRECTION ( 'NONE',  ( -4.274815082592931898E-19, -0.9999939076577903929, -0.003490651415223739937 ) ) ;
#108423=FACE_OUTER_BOUND ( 'NONE', #38065, .T. ) ;
#108424=DIRECTION ( 'NONE',  ( 0.000000000000000000, 0.000000000000000000, -1.000000000000000000 ) ) ;
#108425=ADVANCED_FACE ( 'NONE', ( #55173 ), #82191, .T. ) ;
#108426=CARTESIAN_POINT ( 'NONE',  ( 11.64999999999990798, 12.50000000000000000, 7.253104124594885960 ) ) ;
#108427=CARTESIAN_POINT ( 'NONE',  ( 17.99892161670943125, 2.500000000000000444, -4.934975022999350536 ) ) ;
#108428=LINE ( 'NONE', #10240, #42839 ) ;
#108429=DIRECTION ( 'NONE',  ( 0.000000000000000000, 0.000000000000000000, 1.000000000000000000 ) ) ;
#108430=FACE_OUTER_BOUND ( 'NONE', #122470, .T. ) ;
#108431=AXIS2_PLACEMENT_3D ( 'NONE', #70926, #129228, #892 ) ;
#108432=ORIENTED_EDGE ( 'NONE', *, *, #56839, .T. ) ;
#108433=AXIS2_PLACEMENT_3D ( 'NONE', #10986, #43077, #33246 ) ;
#108434=FACE_OUTER_BOUND ( 'NONE', #27721, .T. ) ;
#108435=LINE ( 'NONE', #77680, #12410 ) ;
#108436=LINE ( 'NONE', #22660, #97637 ) ;
#108437=EDGE_CURVE ( 'NONE', #87221, #108784, #119737, .T. ) ;
#108439=DIRECTION ( 'NONE',  ( -0.000000000000000000, -1.000000000000000000, -0.000000000000000000 ) ) ;
#108440=CONICAL_SURFACE ( 'NONE', #26986, 0.1000000000000002554, 0.003490658503988666988 ) ;
#108441=ORIENTED_EDGE ( 'NONE', *, *, #42967, .F. ) ;
#108442=CIRCLE ( 'NONE', #29052, 0.1000000000000002554 ) ;
#108443=CARTESIAN_POINT ( 'NONE',  ( -2.100000000000033396, 2.500000000000000000, -5.022947341949754119 ) ) ;
#108444=VECTOR ( 'NONE', #8264, 1000.000000000000000 ) ;
#108445=CARTESIAN_POINT ( 'NONE',  ( 5.449999999999936229, 12.50000000000000000, 6.560283801567334372 ) ) ;
#108446=DIRECTION ( 'NONE',  ( 0.000000000000000000, 1.000000000000000000, 0.000000000000000000 ) ) ;
#108447=ORIENTED_EDGE ( 'NONE', *, *, #51437, .T. ) ;
#108448=AXIS2_PLACEMENT_3D ( 'NONE', #94630, #23312, #54696 ) ;
#108449=ORIENTED_EDGE ( 'NONE', *, *, #112931, .F. ) ;
#108450=DIRECTION ( 'NONE',  ( 0.000000000000000000, 0.000000000000000000, 1.000000000000000000 ) ) ;
#108451=CONICAL_SURFACE ( 'NONE', #2028, 0.1000000000000002554, 0.003490658503988666988 ) ;
#108452=EDGE_CURVE ( 'NONE', #62906, #69160, #23598, .T. ) ;
#108453=VERTEX_POINT ( 'NONE', #25062 ) ;
#108454=ORIENTED_EDGE ( 'NONE', *, *, #72646, .F. ) ;
#108456=DIRECTION ( 'NONE',  ( -0.000000000000000000, -1.000000000000000000, -0.000000000000000000 ) ) ;
#108457=EDGE_CURVE ( 'NONE', #112742, #109968, #52850, .T. ) ;
#108458=CARTESIAN_POINT ( 'NONE',  ( 4.349999999999941025, 2.500000000000000000, -1.718653347947326049 ) ) ;
#108459=CARTESIAN_POINT ( 'NONE',  ( -11.24999999999996270, 12.50000000000000000, 2.165063509461097713 ) ) ;
#108460=CARTESIAN_POINT ( 'NONE',  ( -11.64999999999999680, 2.500000000000000000, -7.088010851410849966 ) ) ;
#108461=AXIS2_PLACEMENT_3D ( 'NONE', #46728, #94529, #96450 ) ;
#108462=EDGE_LOOP ( 'NONE', ( #52999, #59455 ) ) ;
#108463=FACE_OUTER_BOUND ( 'NONE', #72965, .T. ) ;
#108464=ORIENTED_EDGE ( 'NONE', *, *, #68620, .T. ) ;
#108465=AXIS2_PLACEMENT_3D ( 'NONE', #88465, #128433, #39410 ) ;
#108466=CARTESIAN_POINT ( 'NONE',  ( -4.400000000000025224, 2.500000000000000000, 3.983716857408420076 ) ) ;
#108467=CARTESIAN_POINT ( 'NONE',  ( 21.24754738303277080, -0.7337760880902398641, -4.182111650399356506 ) ) ;
#108468=FACE_OUTER_BOUND ( 'NONE', #18371, .T. ) ;
#108469=DIRECTION ( 'NONE',  ( 0.000000000000000000, 0.000000000000000000, 1.000000000000000000 ) ) ;
#108470=ADVANCED_FACE ( 'NONE', ( #75439 ), #2760, .T. ) ;
#108471=DIRECTION ( 'NONE',  ( -0.000000000000000000, -1.000000000000000000, -0.000000000000000000 ) ) ;
#108472=ORIENTED_EDGE ( 'NONE', *, *, #94092, .F. ) ;
#108473=CIRCLE ( 'NONE', #89702, 0.09999999999999982514 ) ;
#108474=ORIENTED_EDGE ( 'NONE', *, *, #41722, .F. ) ;
#108475=ORIENTED_EDGE ( 'NONE', *, *, #73353, .T. ) ;
#108476=ORIENTED_EDGE ( 'NONE', *, *, #105591, .T. ) ;
#108477=EDGE_LOOP ( 'NONE', ( #18161, #65425 ) ) ;
#108478=CARTESIAN_POINT ( 'NONE',  ( -1.250000000000037526, 12.50000000000000000, -1.472243186433550122 ) ) ;
#108479=LINE ( 'NONE', #28654, #68659 ) ;
#108480=ADVANCED_FACE ( 'NONE', ( #95742 ), #13115, .T. ) ;
#108481=DIRECTION ( 'NONE',  ( -0.000000000000000000, -1.000000000000000000, -0.000000000000000000 ) ) ;
#108482=FACE_BOUND ( 'NONE', #68942, .T. ) ;
#108483=DIRECTION ( 'NONE',  ( 0.000000000000000000, 0.000000000000000000, 1.000000000000000000 ) ) ;
#108484=CARTESIAN_POINT ( 'NONE',  ( 3.949999999999942446, 2.500000000000000000, -2.511473670974877948 ) ) ;
#108485=CIRCLE ( 'NONE', #52070, 0.1000000000000000056 ) ;
#108486=DIRECTION ( 'NONE',  ( 0.000000000000000000, -0.9999939076577903929, 0.003490651415223739937 ) ) ;
#108487=CARTESIAN_POINT ( 'NONE',  ( 0.7999999999999553024, 2.500000000000000000, -4.330127018922201643 ) ) ;
#108488=AXIS2_PLACEMENT_3D ( 'NONE', #55664, #95597, #5899 ) ;
#108490=DIRECTION ( 'NONE',  ( 0.000000000000000000, 1.000000000000000000, 0.000000000000000000 ) ) ;
#108491=AXIS2_PLACEMENT_3D ( 'NONE', #93264, #3586, #43533 ) ;
#108492=CARTESIAN_POINT ( 'NONE',  ( -12.49999999999999289, 12.50000000000000000, 5.088040615133786027 ) ) ;
#108493=FACE_OUTER_BOUND ( 'NONE', #75367, .T. ) ;
#108494=ADVANCED_FACE ( 'NONE', ( #125827 ), #7341, .T. ) ;
#108495=AXIS2_PLACEMENT_3D ( 'NONE', #43270, #93641, #71401 ) ;
#108496=AXIS2_PLACEMENT_3D ( 'NONE', #64697, #94808, #35259 ) ;
#108497=ORIENTED_EDGE ( 'NONE', *, *, #23495, .F. ) ;
#108498=VERTEX_POINT ( 'NONE', #16510 ) ;
#108499=VERTEX_POINT ( 'NONE', #95100 ) ;
#108500=VERTEX_POINT ( 'NONE', #87191 ) ;
#108501=CARTESIAN_POINT ( 'NONE',  ( 10.44999999999991402, 2.500000000000000000, -2.265063509461101798 ) ) ;
#108502=AXIS2_PLACEMENT_3D ( 'NONE', #110291, #40937, #78921 ) ;
#108503=DIRECTION ( 'NONE',  ( 0.000000000000000000, 1.000000000000000000, 0.000000000000000000 ) ) ;
#108504=FACE_BOUND ( 'NONE', #68752, .T. ) ;
#108505=DIRECTION ( 'NONE',  ( -0.000000000000000000, -1.000000000000000000, -0.000000000000000000 ) ) ;
#108506=EDGE_CURVE ( 'NONE', #45092, #31883, #71722, .T. ) ;
#108507=AXIS2_PLACEMENT_3D ( 'NONE', #81695, #50313, #90213 ) ;
#108508=VERTEX_POINT ( 'NONE', #27619 ) ;
#108509=ADVANCED_FACE ( 'NONE', ( #107494 ), #96742, .T. ) ;
#108510=DIRECTION ( 'NONE',  ( -0.000000000000000000, 1.000000000000000000, -0.000000000000000000 ) ) ;
#108511=CARTESIAN_POINT ( 'NONE',  ( -12.49999999999999467, 2.500000000000000000, -3.637306695894647390 ) ) ;
#108512=EDGE_CURVE ( 'NONE', #8819, #83265, #9011, .T. ) ;
#108513=CARTESIAN_POINT ( 'NONE',  ( 3.749999999999944045, 2.500000000000000000, -7.188010851410854052 ) ) ;
#108514=EDGE_CURVE ( 'NONE', #62002, #119406, #117274, .T. ) ;
#108515=CARTESIAN_POINT ( 'NONE',  ( -9.800000000000007816, 2.500000000000000000, -3.983716857408421852 ) ) ;
#108516=ADVANCED_FACE ( 'NONE', ( #7986 ), #75918, .T. ) ;
#108517=EDGE_LOOP ( 'NONE', ( #26674, #4272 ) ) ;
#108518=CARTESIAN_POINT ( 'NONE',  ( -6.650000000000019007, 2.500000000000000000, -1.372243186433550033 ) ) ;
#108519=VERTEX_POINT ( 'NONE', #38112 ) ;
#108520=ADVANCED_FACE ( 'NONE', ( #25701 ), #117658, .T. ) ;
#108521=EDGE_LOOP ( 'NONE', ( #45622, #50475 ) ) ;
#108522=AXIS2_PLACEMENT_3D ( 'NONE', #58480, #49956, #49312 ) ;
#108523=DIRECTION ( 'NONE',  ( -0.000000000000000000, -1.000000000000000000, -0.000000000000000000 ) ) ;
#108524=EDGE_CURVE ( 'NONE', #117711, #94609, #17437, .T. ) ;
#108525=DIRECTION ( 'NONE',  ( 0.000000000000000000, 0.000000000000000000, 1.000000000000000000 ) ) ;
#108526=ORIENTED_EDGE ( 'NONE', *, *, #54934, .F. ) ;
#108527=EDGE_CURVE ( 'NONE', #77475, #90522, #29867, .T. ) ;
#108528=EDGE_CURVE ( 'NONE', #54254, #74055, #98300, .T. ) ;
#108529=CIRCLE ( 'NONE', #58379, 0.06509327318403745899 ) ;
#108530=DIRECTION ( 'NONE',  ( 0.000000000000000000, -0.9999939076577903929, 0.003490651415223739937 ) ) ;
#108531=EDGE_CURVE ( 'NONE', #108784, #87221, #88435, .T. ) ;
#108532=AXIS2_PLACEMENT_3D ( 'NONE', #97486, #77834, #58852 ) ;
#108533=CARTESIAN_POINT ( 'NONE',  ( 8.349999999999923261, 12.50000000000000000, 2.922977105672686982 ) ) ;
#108534=VERTEX_POINT ( 'NONE', #30886 ) ;
#108535=CARTESIAN_POINT ( 'NONE',  ( -6.900000000000015454, 12.50000000000000000, 4.741630453620009789 ) ) ;
#108537=CARTESIAN_POINT ( 'NONE',  ( 4.999999999999969802, 2.500000000000000000, 4.330127018922196314 ) ) ;
#108538=EDGE_CURVE ( 'NONE', #16823, #32813, #51162, .T. ) ;
#108540=ORIENTED_EDGE ( 'NONE', *, *, #97120, .F. ) ;
#108541=DIRECTION ( 'NONE',  ( -0.000000000000000000, 1.000000000000000000, -0.000000000000000000 ) ) ;
#108542=FACE_BOUND ( 'NONE', #81140, .T. ) ;
#108543=AXIS2_PLACEMENT_3D ( 'NONE', #70430, #118886, #61914 ) ;
#108544=CIRCLE ( 'NONE', #12393, 0.09999999999999982514 ) ;
#108545=ORIENTED_EDGE ( 'NONE', *, *, #59530, .T. ) ;
#108547=VERTEX_POINT ( 'NONE', #70783 ) ;
#108548=DIRECTION ( 'NONE',  ( 0.000000000000000000, -0.000000000000000000, 1.000000000000000000 ) ) ;
#108549=DIRECTION ( 'NONE',  ( -0.000000000000000000, -1.000000000000000000, -0.000000000000000000 ) ) ;
#108550=DIRECTION ( 'NONE',  ( 0.000000000000000000, 0.000000000000000000, 1.000000000000000000 ) ) ;
#108551=DIRECTION ( 'NONE',  ( -4.274815082592931898E-19, -0.9999939076577903929, -0.003490651415223739937 ) ) ;
#108553=AXIS2_PLACEMENT_3D ( 'NONE', #124603, #95141, #123938 ) ;
#108554=VERTEX_POINT ( 'NONE', #50495 ) ;
#108555=ORIENTED_EDGE ( 'NONE', *, *, #73669, .T. ) ;
#108556=CIRCLE ( 'NONE', #43827, 0.06509327318403745899 ) ;
#108557=EDGE_LOOP ( 'NONE', ( #7296, #117632 ) ) ;
#108558=LINE ( 'NONE', #107262, #60144 ) ;
#108559=AXIS2_PLACEMENT_3D ( 'NONE', #38132, #37501, #38809 ) ;
#108560=CARTESIAN_POINT ( 'NONE',  ( -12.09999999999999609, 12.50000000000000000, -0.06509327318403569651 ) ) ;
#108561=DIRECTION ( 'NONE',  ( -4.274815082592931898E-19, -0.9999939076577903929, -0.003490651415223739937 ) ) ;
#108562=VERTEX_POINT ( 'NONE', #30243 ) ;
#108563=ORIENTED_EDGE ( 'NONE', *, *, #59893, .F. ) ;
#108564=EDGE_LOOP ( 'NONE', ( #24304, #14222 ) ) ;
#108565=DIRECTION ( 'NONE',  ( 0.000000000000000000, 1.000000000000000000, 0.000000000000000000 ) ) ;
#108566=CARTESIAN_POINT ( 'NONE',  ( -1.700000000000034817, 2.500000000000000000, -4.230127018922201998 ) ) ;
#108568=DIRECTION ( 'NONE',  ( 0.000000000000000000, 1.000000000000000000, 0.000000000000000000 ) ) ;
#108569=DIRECTION ( 'NONE',  ( -4.274815082592931898E-19, -0.9999939076577903929, -0.003490651415223739937 ) ) ;
#108570=CARTESIAN_POINT ( 'NONE',  ( -10.40000000000000213, 12.50000000000000000, -4.330127018922197202 ) ) ;
#108571=DIRECTION ( 'NONE',  ( 0.000000000000000000, 0.000000000000000000, -1.000000000000000000 ) ) ;
#108572=VECTOR ( 'NONE', #127238, 1000.000000000000000 ) ;
#108573=DIRECTION ( 'NONE',  ( 0.000000000000000000, 1.000000000000000000, 0.000000000000000000 ) ) ;
#108574=DIRECTION ( 'NONE',  ( 0.000000000000000000, 0.000000000000000000, 1.000000000000000000 ) ) ;
#108575=EDGE_LOOP ( 'NONE', ( #1458, #11454 ) ) ;
#108576=ORIENTED_EDGE ( 'NONE', *, *, #88300, .T. ) ;
#108577=ADVANCED_FACE ( 'NONE', ( #1394 ), #73762, .T. ) ;
#108578=DIRECTION ( 'NONE',  ( -4.274815082592931898E-19, -0.9999939076577903929, -0.003490651415223739937 ) ) ;
#108579=ADVANCED_FACE ( 'NONE', ( #28943 ), #94697, .T. ) ;
#108580=CARTESIAN_POINT ( 'NONE',  ( 2.899999999999946620, 2.500000000000000000, -5.022947341949754119 ) ) ;
#108581=ORIENTED_EDGE ( 'NONE', *, *, #85896, .T. ) ;
#108582=ORIENTED_EDGE ( 'NONE', *, *, #31682, .F. ) ;
#108584=DIRECTION ( 'NONE',  ( 0.000000000000000000, 0.000000000000000000, 1.000000000000000000 ) ) ;
#108585=VECTOR ( 'NONE', #113404, 1000.000000000000000 ) ;
#108586=DIRECTION ( 'NONE',  ( 0.000000000000000000, -0.9999939076577903929, 0.003490651415223739937 ) ) ;
#108587=EDGE_CURVE ( 'NONE', #123389, #56994, #38779, .T. ) ;
#108588=CARTESIAN_POINT ( 'NONE',  ( 9.599999999999914380, 12.50000000000000000, -4.330127018922201643 ) ) ;
#108589=CARTESIAN_POINT ( 'NONE',  ( -14.19999999999998685, 12.50000000000000000, -1.084202172485504434E-16 ) ) ;
#108590=CARTESIAN_POINT ( 'NONE',  ( -11.64999999999999680, 2.500000000000000000, -7.088010851410849966 ) ) ;
#108591=DIRECTION ( 'NONE',  ( 0.000000000000000000, 0.000000000000000000, -1.000000000000000000 ) ) ;
#108592=AXIS2_PLACEMENT_3D ( 'NONE', #119333, #69592, #100987 ) ;
#108593=DIRECTION ( 'NONE',  ( -0.000000000000000000, -1.000000000000000000, -0.000000000000000000 ) ) ;
#108594=ORIENTED_EDGE ( 'NONE', *, *, #994, .F. ) ;
#108595=CONICAL_SURFACE ( 'NONE', #50044, 0.1000000000000002554, 0.003490658503988666988 ) ;
#108596=ORIENTED_EDGE ( 'NONE', *, *, #382, .T. ) ;
#108598=AXIS2_PLACEMENT_3D ( 'NONE', #25774, #26431, #57168 ) ;
#108599=ORIENTED_EDGE ( 'NONE', *, *, #85064, .F. ) ;
#108600=ORIENTED_EDGE ( 'NONE', *, *, #30653, .T. ) ;
#108601=CARTESIAN_POINT ( 'NONE',  ( 4.349999999999939249, 2.500000000000000000, 2.411473670974873862 ) ) ;
#108602=DIRECTION ( 'NONE',  ( -0.000000000000000000, -1.000000000000000000, -0.000000000000000000 ) ) ;
#108603=EDGE_LOOP ( 'NONE', ( #58836, #69242 ) ) ;
#108604=DIRECTION ( 'NONE',  ( 0.000000000000000000, 0.000000000000000000, 1.000000000000000000 ) ) ;
#108605=CARTESIAN_POINT ( 'NONE',  ( 10.84999999999991260, 2.500000000000000000, -2.857883832488653741 ) ) ;
#108606=DIRECTION ( 'NONE',  ( -0.000000000000000000, 1.000000000000000000, -0.000000000000000000 ) ) ;
#108607=CARTESIAN_POINT ( 'NONE',  ( -1.250000000000037526, 12.50000000000000000, -1.407149913249512663 ) ) ;
#108608=ORIENTED_EDGE ( 'NONE', *, *, #63892, .T. ) ;
#108609=CARTESIAN_POINT ( 'NONE',  ( 9.149999999999916866, 2.500000000000000000, -1.572243186433550211 ) ) ;
#108610=DIRECTION ( 'NONE',  ( 0.000000000000000000, -0.000000000000000000, 1.000000000000000000 ) ) ;
#108611=ADVANCED_FACE ( 'NONE', ( #68199 ), #50798, .T. ) ;
#108612=ORIENTED_EDGE ( 'NONE', *, *, #32851, .T. ) ;
#108613=ORIENTED_EDGE ( 'NONE', *, *, #28854, .F. ) ;
#108614=ORIENTED_EDGE ( 'NONE', *, *, #27658, .T. ) ;
#108615=AXIS2_PLACEMENT_3D ( 'NONE', #38855, #17882, #68268 ) ;
#108616=ORIENTED_EDGE ( 'NONE', *, *, #124651, .T. ) ;
#108617=DIRECTION ( 'NONE',  ( 0.000000000000000000, 1.000000000000000000, 0.000000000000000000 ) ) ;
#108618=CARTESIAN_POINT ( 'NONE',  ( -2.100000000000033840, 12.50000000000000000, 5.088040615133786027 ) ) ;
#108619=AXIS2_PLACEMENT_3D ( 'NONE', #67862, #58066, #8292 ) ;
#108620=ADVANCED_FACE ( 'NONE', ( #48579 ), #77981, .T. ) ;
#108621=ORIENTED_EDGE ( 'NONE', *, *, #65832, .F. ) ;
#108622=DIRECTION ( 'NONE',  ( -0.000000000000000000, -1.000000000000000000, -0.000000000000000000 ) ) ;
#108623=CARTESIAN_POINT ( 'NONE',  ( 5.599999999999934808, 12.50000000000000000, -4.676537180435978769 ) ) ;
#108624=CARTESIAN_POINT ( 'NONE',  ( 14.79999999999989413, 2.500000000000000000, -0.2464101615137782308 ) ) ;
#108625=DIRECTION ( 'NONE',  ( 0.000000000000000000, 0.000000000000000000, -1.000000000000000000 ) ) ;
#108626=ADVANCED_FACE ( 'NONE', ( #39423 ), #32034, .T. ) ;
#108627=CIRCLE ( 'NONE', #12392, 0.06509327318403741736 ) ;
#108628=AXIS2_PLACEMENT_3D ( 'NONE', #23248, #35038, #114848 ) ;
#108629=VERTEX_POINT ( 'NONE', #110700 ) ;
#108630=DIRECTION ( 'NONE',  ( -0.000000000000000000, 1.000000000000000000, -0.000000000000000000 ) ) ;
#108631=ORIENTED_EDGE ( 'NONE', *, *, #99654, .F. ) ;
#108632=ORIENTED_EDGE ( 'NONE', *, *, #57240, .F. ) ;
#108633=DIRECTION ( 'NONE',  ( 0.000000000000000000, 0.000000000000000000, -1.000000000000000000 ) ) ;
#108634=EDGE_CURVE ( 'NONE', #86589, #6482, #111413, .T. ) ;
#108635=CARTESIAN_POINT ( 'NONE',  ( 4.799999999999937650, 12.50000000000000000, -0.4115034346978156399 ) ) ;
#108636=FACE_BOUND ( 'NONE', #68845, .T. ) ;
#108638=DIRECTION ( 'NONE',  ( 0.000000000000000000, 0.000000000000000000, -1.000000000000000000 ) ) ;
#108640=CARTESIAN_POINT ( 'NONE',  ( -1.050000000000038680, 12.50000000000000000, 6.906693963081109722 ) ) ;
#108641=AXIS2_PLACEMENT_3D ( 'NONE', #68200, #18463, #40710 ) ;
#108642=CONICAL_SURFACE ( 'NONE', #27089, 0.1000000000000000472, 0.003490658503988666988 ) ;
#108643=VERTEX_POINT ( 'NONE', #78696 ) ;
#108644=DIRECTION ( 'NONE',  ( 0.000000000000000000, -0.000000000000000000, 1.000000000000000000 ) ) ;
#108645=LINE ( 'NONE', #68074, #32301 ) ;
#108646=CARTESIAN_POINT ( 'NONE',  ( 4.149999999999939959, 12.50000000000000000, 1.537336459617582918 ) ) ;
#108647=DIRECTION ( 'NONE',  ( -0.000000000000000000, -1.000000000000000000, -0.000000000000000000 ) ) ;
#108648=ORIENTED_EDGE ( 'NONE', *, *, #91523, .T. ) ;
#108649=AXIS2_PLACEMENT_3D ( 'NONE', #107345, #74666, #17671 ) ;
#108650=DIRECTION ( 'NONE',  ( 0.000000000000000000, -0.000000000000000000, 1.000000000000000000 ) ) ;
#108651=DIRECTION ( 'NONE',  ( 0.000000000000000000, 1.000000000000000000, 0.000000000000000000 ) ) ;
#108652=CIRCLE ( 'NONE', #116957, 0.06509327318403745899 ) ;
#108653=ORIENTED_EDGE ( 'NONE', *, *, #25077, .F. ) ;
#108654=ORIENTED_EDGE ( 'NONE', *, *, #22842, .F. ) ;
#108655=FACE_OUTER_BOUND ( 'NONE', #14670, .T. ) ;
#108656=DIRECTION ( 'NONE',  ( -0.000000000000000000, -1.000000000000000000, -0.000000000000000000 ) ) ;
#108657=FACE_BOUND ( 'NONE', #52672, .T. ) ;
#108658=CARTESIAN_POINT ( 'NONE',  ( 7.699999999999922018, 2.500000000000000000, 0.3464101615137735735 ) ) ;
#108659=EDGE_CURVE ( 'NONE', #90797, #36770, #118590, .T. ) ;
#108660=ORIENTED_EDGE ( 'NONE', *, *, #99043, .F. ) ;
#108661=CARTESIAN_POINT ( 'NONE',  ( 4.999999999999933387, 2.500000000000000000, 5.022947341949748790 ) ) ;
#108662=ORIENTED_EDGE ( 'NONE', *, *, #70563, .F. ) ;
#108663=( BOUNDED_SURFACE ( )  B_SPLINE_SURFACE ( 3, 2, ( 
 ( #27981, #65313, #94791 ),
 ( #124896, #17499, #116351 ),
 ( #107174, #35874, #77086 ),
 ( #77709, #115052, #116985 ),
 ( #86238, #35242, #96706 ),
 ( #27316, #67221, #57447 ),
 ( #105251, #36534, #105901 ),
 ( #45065, #76444, #87536 ),
 ( #97365, #26695, #5740 ),
 ( #67900, #84964, #7679 ),
 ( #46991, #47627, #127477 ),
 ( #25386, #65972, #117618 ) ),
 .UNSPECIFIED., .F., .F., .F. ) 
 B_SPLINE_SURFACE_WITH_KNOTS ( ( 4, 2, 2, 2, 2, 4 ),
 ( 3, 3 ),
 ( -5.075233897142896741E-05, 0.01652955890756899540, 0.03310987015410941925, 0.04969018140064984657, 0.05798033702392006022, 0.06627049264719027388 ),
 ( 0.000000000000000000, 1.000000000000000000 ),
 .UNSPECIFIED. ) 
 GEOMETRIC_REPRESENTATION_ITEM ( )  RATIONAL_B_SPLINE_SURFACE ( (
 ( 1.000000000000000000, 1.000000000000000000, 1.000000000000000000),
 ( 1.000000000000000000, 0.9999962913215033611, 1.000000000000000000),
 ( 1.000000000000000000, 0.9967432547760589623, 1.000000000000000000),
 ( 1.000000000000000000, 0.9780629203682255079, 1.000000000000000000),
 ( 1.000000000000000000, 0.9624374449458362735, 1.000000000000000000),
 ( 1.000000000000000000, 0.9156028756809130309, 1.000000000000000000),
 ( 1.000000000000000000, 0.8842425818972232676, 1.000000000000000000),
 ( 1.000000000000000000, 0.8293059173979305809, 1.000000000000000000),
 ( 1.000000000000000000, 0.8097380764759147809, 1.000000000000000000),
 ( 1.000000000000000000, 0.7702514575408279107, 1.000000000000000000),
 ( 1.000000000000000000, 0.7503390841288218871, 1.000000000000000000),
 ( 1.000000000000000000, 0.7318752858502189929, 1.000000000000000000) ) ) 
 REPRESENTATION_ITEM ( '' )  SURFACE ( )  );
#108664=VERTEX_POINT ( 'NONE', #83198 ) ;
#108666=EDGE_CURVE ( 'NONE', #81572, #8476, #105160, .T. ) ;
#108668=EDGE_CURVE ( 'NONE', #73062, #37904, #3337, .T. ) ;
#108669=VERTEX_POINT ( 'NONE', #13784 ) ;
#108670=LINE ( 'NONE', #18989, #17559 ) ;
#108671=DIRECTION ( 'NONE',  ( 0.000000000000000000, 1.000000000000000000, 0.000000000000000000 ) ) ;
#108672=EDGE_CURVE ( 'NONE', #88690, #74641, #91715, .T. ) ;
#108673=ADVANCED_FACE ( 'NONE', ( #24261 ), #90585, .T. ) ;
#108674=CARTESIAN_POINT ( 'NONE',  ( -8.150000000000014566, 12.50000000000000000, -6.148780366869520897 ) ) ;
#108675=AXIS2_PLACEMENT_3D ( 'NONE', #86980, #126269, #34684 ) ;
#108676=ADVANCED_FACE ( 'NONE', ( #121813 ), #6938, .T. ) ;
#108677=DIRECTION ( 'NONE',  ( 0.000000000000000000, -0.9999939076577903929, 0.003490651415223739937 ) ) ;
#108678=EDGE_LOOP ( 'NONE', ( #10349, #21409, #122662, #111572 ) ) ;
#108679=FACE_OUTER_BOUND ( 'NONE', #11608, .T. ) ;
#108680=AXIS2_PLACEMENT_3D ( 'NONE', #50824, #41022, #12163 ) ;
#108681=CIRCLE ( 'NONE', #52262, 0.1000000000000002554 ) ;
#108682=ADVANCED_FACE ( 'NONE', ( #53723 ), #44627, .T. ) ;
#108683=CARTESIAN_POINT ( 'NONE',  ( -3.750000000000026201, 2.500000000000000000, 5.802370205355744659 ) ) ;
#108685=DIRECTION ( 'NONE',  ( 0.000000000000000000, 0.000000000000000000, 1.000000000000000000 ) ) ;
#108686=VERTEX_POINT ( 'NONE', #93653 ) ;
#108687=ORIENTED_EDGE ( 'NONE', *, *, #89777, .F. ) ;
#108688=CARTESIAN_POINT ( 'NONE',  ( -12.09999999999999609, 2.500000000000000000, -3.537306695894647302 ) ) ;
#108689=EDGE_CURVE ( 'NONE', #47413, #100917, #2857, .T. ) ;
#108690=ORIENTED_EDGE ( 'NONE', *, *, #45358, .T. ) ;
#108691=DIRECTION ( 'NONE',  ( 0.000000000000000000, -0.9999939076577903929, 0.003490651415223739937 ) ) ;
#108693=AXIS2_PLACEMENT_3D ( 'NONE', #113303, #113956, #94969 ) ;
#108694=DIRECTION ( 'NONE',  ( 0.000000000000000000, 0.000000000000000000, -1.000000000000000000 ) ) ;
#108695=CARTESIAN_POINT ( 'NONE',  ( -3.950000000000024603, 12.50000000000000000, 1.883746621131358934 ) ) ;
#108696=CARTESIAN_POINT ( 'NONE',  ( 6.899999999999928413, 2.500000000000000000, 4.676537180435972552 ) ) ;
#108697=ORIENTED_EDGE ( 'NONE', *, *, #45744, .T. ) ;
#108698=CARTESIAN_POINT ( 'NONE',  ( -14.79999999999998295, 2.500000000000000000, -0.3464101615137760715 ) ) ;
#108699=DIRECTION ( 'NONE',  ( 0.000000000000000000, -0.9999939076577903929, 0.003490651415223739937 ) ) ;
#108700=CARTESIAN_POINT ( 'NONE',  ( 81.97642828244310920, 3.858501901686324675, -6.173828276686423422 ) ) ;
#108702=CARTESIAN_POINT ( 'NONE',  ( 8.949999999999915801, 2.500000000000000000, -1.818653347947326138 ) ) ;
#108703=CARTESIAN_POINT ( 'NONE',  ( 7.499999999999925393, 2.500000000000000000, -3.737306695894649700 ) ) ;
#108704=ORIENTED_EDGE ( 'NONE', *, *, #114097, .F. ) ;
#108705=ORIENTED_EDGE ( 'NONE', *, *, #116206, .T. ) ;
#108706=DIRECTION ( 'NONE',  ( 0.000000000000000000, 0.000000000000000000, -1.000000000000000000 ) ) ;
#108707=ORIENTED_EDGE ( 'NONE', *, *, #57557, .T. ) ;
#108708=CARTESIAN_POINT ( 'NONE',  ( -15.39999999999997904, 2.500000000000000000, 0.000000000000000000 ) ) ;
#108709=ORIENTED_EDGE ( 'NONE', *, *, #2584, .T. ) ;
#108710=ORIENTED_EDGE ( 'NONE', *, *, #25320, .T. ) ;
#108711=VERTEX_POINT ( 'NONE', #72724 ) ;
#108712=FACE_OUTER_BOUND ( 'NONE', #36059, .T. ) ;
#108713=CARTESIAN_POINT ( 'NONE',  ( 2.899999999999943956, 2.500000000000000000, 4.430127018922196847 ) ) ;
#108714=AXIS2_PLACEMENT_3D ( 'NONE', #129178, #87276, #127226 ) ;
#108715=FACE_OUTER_BOUND ( 'NONE', #30488, .T. ) ;
#108716=CARTESIAN_POINT ( 'NONE',  ( -10.65000000000000213, 2.500000000000000000, 6.148780366869520009 ) ) ;
#108717=DIRECTION ( 'NONE',  ( 0.000000000000000000, 0.000000000000000000, -1.000000000000000000 ) ) ;
#108718=CARTESIAN_POINT ( 'NONE',  ( 5.399999999999936406, 2.500000000000000000, -5.122947341949753763 ) ) ;
#108719=FACE_OUTER_BOUND ( 'NONE', #86724, .T. ) ;
#108720=DIRECTION ( 'NONE',  ( 0.000000000000000000, -0.000000000000000000, 1.000000000000000000 ) ) ;
#108721=CIRCLE ( 'NONE', #62852, 0.06509327318403745899 ) ;
#108722=EDGE_LOOP ( 'NONE', ( #66725, #88545 ) ) ;
#108723=ORIENTED_EDGE ( 'NONE', *, *, #110394, .T. ) ;
#108724=EDGE_CURVE ( 'NONE', #61381, #94776, #19586, .T. ) ;
#108725=DIRECTION ( 'NONE',  ( -0.000000000000000000, 1.000000000000000000, -0.000000000000000000 ) ) ;
#108726=VERTEX_POINT ( 'NONE', #31509 ) ;
#108727=EDGE_LOOP ( 'NONE', ( #127251, #10156, #114116, #22002 ) ) ;
#108728=DIRECTION ( 'NONE',  ( 0.000000000000000000, -0.9999939076577903929, 0.003490651415223739937 ) ) ;
#108729=AXIS2_PLACEMENT_3D ( 'NONE', #29959, #6560, #89512 ) ;
#108730=ADVANCED_FACE ( 'NONE', ( #121175 ), #86381, .T. ) ;
#108731=AXIS2_PLACEMENT_3D ( 'NONE', #106828, #6050, #17136 ) ;
#108732=CARTESIAN_POINT ( 'NONE',  ( -11.25000000000000000, 2.500000000000000000, 2.857883832488649301 ) ) ;
#108733=AXIS2_PLACEMENT_3D ( 'NONE', #83219, #123139, #34120 ) ;
#108734=CARTESIAN_POINT ( 'NONE',  ( 5.799999999999933209, 12.50000000000000000, -2.385244779468109755E-15 ) ) ;
#108735=CARTESIAN_POINT ( 'NONE',  ( 4.549999999999935874, 2.500000000000000000, 6.395190528383296602 ) ) ;
#108736=CARTESIAN_POINT ( 'NONE',  ( 1.699999999999950218, 2.500000000000000000, 4.330127018922196314 ) ) ;
#108738=CIRCLE ( 'NONE', #121350, 0.06509327318403745899 ) ;
#108739=ORIENTED_EDGE ( 'NONE', *, *, #51797, .T. ) ;
#108740=DIRECTION ( 'NONE',  ( 0.000000000000000000, -0.000000000000000000, 1.000000000000000000 ) ) ;
#108741=ORIENTED_EDGE ( 'NONE', *, *, #73045, .T. ) ;
#108742=CARTESIAN_POINT ( 'NONE',  ( 8.749999999999923617, 2.500000000000000000, 1.472243186433545459 ) ) ;
#108743=AXIS2_PLACEMENT_3D ( 'NONE', #128322, #27495, #107371 ) ;
#108744=VERTEX_POINT ( 'NONE', #61626 ) ;
#108745=ORIENTED_EDGE ( 'NONE', *, *, #128660, .F. ) ;
#108746=CARTESIAN_POINT ( 'NONE',  ( 1.249999999999953815, 2.500000000000000000, -2.957883832488653830 ) ) ;
#108747=CARTESIAN_POINT ( 'NONE',  ( 5.199999999999935341, 2.500000000000000000, -3.983716857408426293 ) ) ;
#108748=DIRECTION ( 'NONE',  ( 0.000000000000000000, 0.000000000000000000, -1.000000000000000000 ) ) ;
#108749=DIRECTION ( 'NONE',  ( 0.000000000000000000, 0.000000000000000000, -1.000000000000000000 ) ) ;
#108750=DIRECTION ( 'NONE',  ( 0.000000000000000000, 0.000000000000000000, 1.000000000000000000 ) ) ;
#108751=ORIENTED_EDGE ( 'NONE', *, *, #49916, .F. ) ;
#108752=DIRECTION ( 'NONE',  ( -4.274815082592931898E-19, -0.9999939076577903929, -0.003490651415223739937 ) ) ;
#108753=LINE ( 'NONE', #50487, #62056 ) ;
#108754=CARTESIAN_POINT ( 'NONE',  ( 4.999999999999936939, 12.50000000000000000, -0.6928203230275541413 ) ) ;
#108755=CARTESIAN_POINT ( 'NONE',  ( -0.2000000000000404232, 12.50000000000000000, 3.983716857408420964 ) ) ;
#108756=DIRECTION ( 'NONE',  ( -0.000000000000000000, 1.000000000000000000, -0.000000000000000000 ) ) ;
#108757=ADVANCED_FACE ( 'NONE', ( #113278 ), #63552, .T. ) ;
#108758=ORIENTED_EDGE ( 'NONE', *, *, #42961, .T. ) ;
#108759=VERTEX_POINT ( 'NONE', #112649 ) ;
#108760=VECTOR ( 'NONE', #60617, 1000.000000000000000 ) ;
#108761=CARTESIAN_POINT ( 'NONE',  ( 2.099999999999950351, 2.500000000000000000, -4.922947341949753586 ) ) ;
#108762=CIRCLE ( 'NONE', #50293, 0.1000000000000000472 ) ;
#108763=ORIENTED_EDGE ( 'NONE', *, *, #110128, .T. ) ;
#108764=DIRECTION ( 'NONE',  ( -0.000000000000000000, -1.000000000000000000, -0.000000000000000000 ) ) ;
#108765=DIRECTION ( 'NONE',  ( -0.000000000000000000, 1.000000000000000000, -0.000000000000000000 ) ) ;
#108766=EDGE_CURVE ( 'NONE', #17919, #77627, #81875, .T. ) ;
#108767=VECTOR ( 'NONE', #34915, 1000.000000000000000 ) ;
#108768=CIRCLE ( 'NONE', #38106, 0.1000000000000000472 ) ;
#108769=EDGE_CURVE ( 'NONE', #14739, #10534, #27898, .T. ) ;
#108771=DIRECTION ( 'NONE',  ( 0.000000000000000000, 1.000000000000000000, 0.000000000000000000 ) ) ;
#108772=CARTESIAN_POINT ( 'NONE',  ( -5.600000000000020073, 12.50000000000000000, 4.048810130592458201 ) ) ;
#108773=DIRECTION ( 'NONE',  ( 0.000000000000000000, 0.000000000000000000, 1.000000000000000000 ) ) ;
#108774=EDGE_CURVE ( 'NONE', #46669, #36193, #74011, .T. ) ;
#108775=DIRECTION ( 'NONE',  ( 0.000000000000000000, 0.000000000000000000, 1.000000000000000000 ) ) ;
#108776=ORIENTED_EDGE ( 'NONE', *, *, #115236, .T. ) ;
#108777=DIRECTION ( 'NONE',  ( -0.000000000000000000, -1.000000000000000000, -0.000000000000000000 ) ) ;
#108778=EDGE_CURVE ( 'NONE', #92869, #33146, #128267, .T. ) ;
#108779=VERTEX_POINT ( 'NONE', #53083 ) ;
#108780=EDGE_CURVE ( 'NONE', #34969, #89288, #43280, .T. ) ;
#108781=CARTESIAN_POINT ( 'NONE',  ( 24.00483293780993321, 0.9037283375177144196, -4.313967621098822036 ) ) ;
#108782=CARTESIAN_POINT ( 'NONE',  ( -11.69999999999999574, 12.50000000000000000, 4.330127018922196314 ) ) ;
#108783=DIRECTION ( 'NONE',  ( 0.000000000000000000, -0.000000000000000000, 1.000000000000000000 ) ) ;
#108784=VERTEX_POINT ( 'NONE', #3969 ) ;
#108785=DIRECTION ( 'NONE',  ( 0.000000000000000000, 0.000000000000000000, -1.000000000000000000 ) ) ;
#108786=ORIENTED_EDGE ( 'NONE', *, *, #40416, .F. ) ;
#108788=DIRECTION ( 'NONE',  ( -0.000000000000000000, -1.000000000000000000, -0.000000000000000000 ) ) ;
#108789=DIRECTION ( 'NONE',  ( -0.000000000000000000, 1.000000000000000000, -0.000000000000000000 ) ) ;
#108790=ORIENTED_EDGE ( 'NONE', *, *, #67786, .T. ) ;
#108791=CIRCLE ( 'NONE', #54509, 0.06509327318403745899 ) ;
#108792=DIRECTION ( 'NONE',  ( -0.000000000000000000, 1.000000000000000000, -0.000000000000000000 ) ) ;
#108793=AXIS2_PLACEMENT_3D ( 'NONE', #53526, #4382, #44331 ) ;
#108794=DIRECTION ( 'NONE',  ( -0.000000000000000000, -1.000000000000000000, -0.000000000000000000 ) ) ;
#108795=ADVANCED_FACE ( 'NONE', ( #83818 ), #25849, .T. ) ;
#108796=ORIENTED_EDGE ( 'NONE', *, *, #83444, .T. ) ;
#108797=DIRECTION ( 'NONE',  ( -0.000000000000000000, 1.000000000000000000, -0.000000000000000000 ) ) ;
#108798=ORIENTED_EDGE ( 'NONE', *, *, #40603, .T. ) ;
#108799=AXIS2_PLACEMENT_3D ( 'NONE', #21377, #61317, #19437 ) ;
#108800=DIRECTION ( 'NONE',  ( 0.000000000000000000, 0.000000000000000000, 1.000000000000000000 ) ) ;
#108801=EDGE_CURVE ( 'NONE', #124608, #77665, #44550, .T. ) ;
#108802=ORIENTED_EDGE ( 'NONE', *, *, #39285, .T. ) ;
#108803=CARTESIAN_POINT ( 'NONE',  ( -8.350000000000013856, 12.50000000000000000, -6.495190528383297135 ) ) ;
#108804=DIRECTION ( 'NONE',  ( -0.000000000000000000, 1.000000000000000000, -0.000000000000000000 ) ) ;
#108805=EDGE_LOOP ( 'NONE', ( #78176, #111080 ) ) ;
#108806=EDGE_LOOP ( 'NONE', ( #26104, #14634 ) ) ;
#108807=DIRECTION ( 'NONE',  ( -0.000000000000000000, 1.000000000000000000, -0.000000000000000000 ) ) ;
#108808=CARTESIAN_POINT ( 'NONE',  ( -9.550000000000006040, 2.500000000000000000, -2.165063509461101710 ) ) ;
#108809=ORIENTED_EDGE ( 'NONE', *, *, #5073, .T. ) ;
#108810=ADVANCED_FACE ( 'NONE', ( #34750 ), #103113, .T. ) ;
#108811=AXIS2_PLACEMENT_3D ( 'NONE', #106046, #5888, #26843 ) ;
#108812=LINE ( 'NONE', #58456, #69811 ) ;
#108814=CARTESIAN_POINT ( 'NONE',  ( 12.94999999999990337, 2.500000000000000000, 2.165063509461097713 ) ) ;
#108816=DIRECTION ( 'NONE',  ( 0.000000000000000000, 0.000000000000000000, 1.000000000000000000 ) ) ;
#108817=EDGE_CURVE ( 'NONE', #32380, #95927, #101058, .T. ) ;
#108818=DIRECTION ( 'NONE',  ( -0.000000000000000000, 1.000000000000000000, -0.000000000000000000 ) ) ;
#108819=LINE ( 'NONE', #97721, #96486 ) ;
#108820=EDGE_CURVE ( 'NONE', #37294, #78706, #105258, .T. ) ;
#108821=CIRCLE ( 'NONE', #39903, 0.1000000000000002554 ) ;
#108822=ADVANCED_FACE ( 'NONE', ( #74647 ), #97988, .T. ) ;
#108823=ORIENTED_EDGE ( 'NONE', *, *, #17420, .T. ) ;
#108824=EDGE_LOOP ( 'NONE', ( #5803, #5330 ) ) ;
#108825=EDGE_CURVE ( 'NONE', #9410, #86367, #24908, .T. ) ;
#108826=VERTEX_POINT ( 'NONE', #118924 ) ;
#108827=ORIENTED_EDGE ( 'NONE', *, *, #36978, .F. ) ;
#108828=DIRECTION ( 'NONE',  ( 0.000000000000000000, -0.000000000000000000, 1.000000000000000000 ) ) ;
#108829=DIRECTION ( 'NONE',  ( 0.000000000000000000, 1.000000000000000000, 0.000000000000000000 ) ) ;
#108830=DIRECTION ( 'NONE',  ( 0.000000000000000000, 0.000000000000000000, 1.000000000000000000 ) ) ;
#108831=VERTEX_POINT ( 'NONE', #55004 ) ;
#108832=FACE_BOUND ( 'NONE', #56904, .T. ) ;
#108833=ORIENTED_EDGE ( 'NONE', *, *, #79641, .F. ) ;
#108834=CARTESIAN_POINT ( 'NONE',  ( 1.049999999999953637, 2.500000000000000000, -1.818653347947326138 ) ) ;
#108835=CARTESIAN_POINT ( 'NONE',  ( -9.800000000000006040, 12.50000000000000000, 4.741630453620009789 ) ) ;
#108836=ADVANCED_FACE ( 'NONE', ( #48248 ), #15047, .T. ) ;
#108837=EDGE_CURVE ( 'NONE', #73563, #12234, #69161, .T. ) ;
#108838=LINE ( 'NONE', #110775, #70179 ) ;
#108839=EDGE_CURVE ( 'NONE', #53810, #99657, #38387, .T. ) ;
#108840=LINE ( 'NONE', #17886, #120317 ) ;
#108841=CARTESIAN_POINT ( 'NONE',  ( -5.850000000000018296, 2.500000000000000000, 2.857883832488649301 ) ) ;
#108842=DIRECTION ( 'NONE',  ( 0.000000000000000000, 0.000000000000000000, 1.000000000000000000 ) ) ;
#108843=CARTESIAN_POINT ( 'NONE',  ( 2.699999999999947331, 2.500000000000000000, -4.676537180435978769 ) ) ;
#108844=DIRECTION ( 'NONE',  ( 0.000000000000000000, -0.9999939076577903929, 0.003490651415223739937 ) ) ;
#108845=DIRECTION ( 'NONE',  ( 0.000000000000000000, 0.000000000000000000, 1.000000000000000000 ) ) ;
#108846=CARTESIAN_POINT ( 'NONE',  ( 6.049999999999932321, 12.50000000000000000, -1.818653347947326138 ) ) ;
#108847=ORIENTED_EDGE ( 'NONE', *, *, #58159, .T. ) ;
#108848=ORIENTED_EDGE ( 'NONE', *, *, #73509, .F. ) ;
#108849=ORIENTED_EDGE ( 'NONE', *, *, #106943, .F. ) ;
#108850=EDGE_LOOP ( 'NONE', ( #101807, #96010 ) ) ;
#108851=CARTESIAN_POINT ( 'NONE',  ( 3.549999999999943867, 12.50000000000000000, -6.213873640053564351 ) ) ;
#108852=AXIS2_PLACEMENT_3D ( 'NONE', #98915, #69445, #30842 ) ;
#108853=DIRECTION ( 'NONE',  ( -0.000000000000000000, 1.000000000000000000, -0.000000000000000000 ) ) ;
#108854=VECTOR ( 'NONE', #43551, 1000.000000000000000 ) ;
#108855=ORIENTED_EDGE ( 'NONE', *, *, #122127, .T. ) ;
#108856=ORIENTED_EDGE ( 'NONE', *, *, #37712, .T. ) ;
#108857=EDGE_LOOP ( 'NONE', ( #12242, #81104 ) ) ;
#108858=DIRECTION ( 'NONE',  ( 0.000000000000000000, 0.000000000000000000, 1.000000000000000000 ) ) ;
#108859=CARTESIAN_POINT ( 'NONE',  ( -11.05000000000000071, 2.500000000000000000, -2.411473670974874306 ) ) ;
#108861=CARTESIAN_POINT ( 'NONE',  ( -4.350000000000023626, 12.50000000000000000, 1.818653347947321475 ) ) ;
#108862=DIRECTION ( 'NONE',  ( 0.000000000000000000, 1.000000000000000000, 0.000000000000000000 ) ) ;
#108863=LINE ( 'NONE', #19184, #60213 ) ;
#108864=CIRCLE ( 'NONE', #4385, 0.1000000000000002554 ) ;
#108865=CARTESIAN_POINT ( 'NONE',  ( -8.749999999999975131, 12.50000000000000000, -2.099970236277064473 ) ) ;
#108866=VERTEX_POINT ( 'NONE', #28622 ) ;
#108867=CARTESIAN_POINT ( 'NONE',  ( -6.900000000000019007, 12.50000000000000000, -4.676537180435978769 ) ) ;
#108868=VERTEX_POINT ( 'NONE', #75291 ) ;
#108869=ORIENTED_EDGE ( 'NONE', *, *, #28005, .F. ) ;
#108870=EDGE_LOOP ( 'NONE', ( #124130, #74494, #57676, #124493 ) ) ;
#108871=CARTESIAN_POINT ( 'NONE',  ( -0.6500000000000403233, 12.50000000000000000, 6.148780366869520009 ) ) ;
#108872=EDGE_LOOP ( 'NONE', ( #91084, #74907, #100037, #44010 ) ) ;
#108873=EDGE_LOOP ( 'NONE', ( #61613, #56041 ) ) ;
#108874=DIRECTION ( 'NONE',  ( 0.000000000000000000, 0.000000000000000000, -1.000000000000000000 ) ) ;
#108875=EDGE_CURVE ( 'NONE', #86483, #127093, #80135, .T. ) ;
#108876=VECTOR ( 'NONE', #33384, 1000.000000000000000 ) ;
#108877=CARTESIAN_POINT ( 'NONE',  ( -13.09999999999999076, 2.500000000000000000, 3.983716857408420964 ) ) ;
#108878=DIRECTION ( 'NONE',  ( 0.000000000000000000, 0.000000000000000000, 1.000000000000000000 ) ) ;
#108879=DIRECTION ( 'NONE',  ( 0.000000000000000000, 1.000000000000000000, 0.000000000000000000 ) ) ;
#108880=FACE_OUTER_BOUND ( 'NONE', #55040, .T. ) ;
#108881=VERTEX_POINT ( 'NONE', #85749 ) ;
#108882=DIRECTION ( 'NONE',  ( 0.000000000000000000, -0.000000000000000000, 1.000000000000000000 ) ) ;
#108883=AXIS2_PLACEMENT_3D ( 'NONE', #100078, #119703, #30056 ) ;
#108884=AXIS2_PLACEMENT_3D ( 'NONE', #73000, #94561, #22632 ) ;
#108885=EDGE_LOOP ( 'NONE', ( #35841, #110356 ) ) ;
#108886=DIRECTION ( 'NONE',  ( 0.000000000000000000, 0.000000000000000000, -1.000000000000000000 ) ) ;
#108887=EDGE_LOOP ( 'NONE', ( #67204, #66687 ) ) ;
#108888=DIRECTION ( 'NONE',  ( 0.000000000000000000, 0.000000000000000000, -1.000000000000000000 ) ) ;
#108889=CARTESIAN_POINT ( 'NONE',  ( 9.349999999999919709, 12.50000000000000000, -6.083687093685488989 ) ) ;
#108890=EDGE_LOOP ( 'NONE', ( #82142, #28380, #33426, #106689 ) ) ;
#108891=DIRECTION ( 'NONE',  ( -0.000000000000000000, -1.000000000000000000, -0.000000000000000000 ) ) ;
#108892=DIRECTION ( 'NONE',  ( -0.000000000000000000, -1.000000000000000000, -0.000000000000000000 ) ) ;
#108893=ORIENTED_EDGE ( 'NONE', *, *, #31272, .F. ) ;
#108894=AXIS2_PLACEMENT_3D ( 'NONE', #84156, #84805, #74346 ) ;
#108895=AXIS2_PLACEMENT_3D ( 'NONE', #11821, #22947, #21655 ) ;
#108896=CARTESIAN_POINT ( 'NONE',  ( 13.14999999999990088, 12.50000000000000000, 1.818653347947321475 ) ) ;
#108897=ORIENTED_EDGE ( 'NONE', *, *, #109891, .T. ) ;
#108898=ORIENTED_EDGE ( 'NONE', *, *, #23778, .T. ) ;
#108899=CARTESIAN_POINT ( 'NONE',  ( 2.049999999999948308, 2.500000000000000000, 6.395190528383296602 ) ) ;
#108900=CARTESIAN_POINT ( 'NONE',  ( -11.44999999999999751, 12.50000000000000000, 1.818653347947321475 ) ) ;
#108901=CARTESIAN_POINT ( 'NONE',  ( -11.44999999999999751, 2.500000000000000000, 6.148780366869520897 ) ) ;
#108902=DIRECTION ( 'NONE',  ( 0.000000000000000000, 0.000000000000000000, 1.000000000000000000 ) ) ;
#108903=CIRCLE ( 'NONE', #77524, 0.1000000000000000056 ) ;
#108904=VECTOR ( 'NONE', #61327, 1000.000000000000000 ) ;
#108905=DIRECTION ( 'NONE',  ( 0.000000000000000000, 0.000000000000000000, 1.000000000000000000 ) ) ;
#108906=EDGE_LOOP ( 'NONE', ( #120024, #96000 ) ) ;
#108907=LINE ( 'NONE', #19238, #105115 ) ;
#108908=AXIS2_PLACEMENT_3D ( 'NONE', #125398, #35728, #115550 ) ;
#108909=VERTEX_POINT ( 'NONE', #19418 ) ;
#108910=DIRECTION ( 'NONE',  ( 0.000000000000000000, 1.000000000000000000, 0.000000000000000000 ) ) ;
#108911=CARTESIAN_POINT ( 'NONE',  ( -3.100000000000028511, 2.500000000000000000, 0.3464101615137736845 ) ) ;
#108912=ADVANCED_FACE ( 'NONE', ( #5254 ), #75932, .T. ) ;
#108913=ORIENTED_EDGE ( 'NONE', *, *, #89005, .T. ) ;
#108914=AXIS2_PLACEMENT_3D ( 'NONE', #63766, #121382, #44114 ) ;
#108915=AXIS2_PLACEMENT_3D ( 'NONE', #28572, #77656, #117558 ) ;
#108916=EDGE_CURVE ( 'NONE', #31016, #113497, #48844, .T. ) ;
#108917=LINE ( 'NONE', #47445, #97438 ) ;
#108918=CARTESIAN_POINT ( 'NONE',  ( -5.450000000000019718, 2.500000000000000000, 2.265063509461097357 ) ) ;
#108919=CARTESIAN_POINT ( 'NONE',  ( -13.54999999999999005, 12.50000000000000000, -1.818653347947323917 ) ) ;
#108920=DIRECTION ( 'NONE',  ( -0.000000000000000000, -1.000000000000000000, -0.000000000000000000 ) ) ;
#108921=EDGE_CURVE ( 'NONE', #23572, #83529, #96842, .T. ) ;
#108922=DIRECTION ( 'NONE',  ( -0.000000000000000000, -1.000000000000000000, -0.000000000000000000 ) ) ;
#108923=ORIENTED_EDGE ( 'NONE', *, *, #106639, .F. ) ;
#108924=CARTESIAN_POINT ( 'NONE',  ( 13.14999999999989733, 2.500000000000000000, -1.718653347947325827 ) ) ;
#108925=LINE ( 'NONE', #88659, #72337 ) ;
#108926=CARTESIAN_POINT ( 'NONE',  ( 4.199999999999939782, 12.50000000000000000, -2.276824562219559311E-15 ) ) ;
#108927=ADVANCED_FACE ( 'NONE', ( #15715 ), #40442, .T. ) ;
#108929=EDGE_CURVE ( 'NONE', #7665, #7181, #63408, .T. ) ;
#108930=EDGE_LOOP ( 'NONE', ( #68043, #90240 ) ) ;
#108931=CARTESIAN_POINT ( 'NONE',  ( 3.949999999999939782, 12.50000000000000000, 2.511473670974873507 ) ) ;
#108932=ORIENTED_EDGE ( 'NONE', *, *, #43819, .F. ) ;
#108933=ORIENTED_EDGE ( 'NONE', *, *, #76315, .F. ) ;
#108934=DIRECTION ( 'NONE',  ( 0.000000000000000000, 0.000000000000000000, 1.000000000000000000 ) ) ;
#108935=AXIS2_PLACEMENT_3D ( 'NONE', #54625, #94553, #44835 ) ;
#108937=DIRECTION ( 'NONE',  ( 0.000000000000000000, -0.000000000000000000, 1.000000000000000000 ) ) ;
#108938=CARTESIAN_POINT ( 'NONE',  ( 3.949999999999941558, 12.50000000000000000, -6.083687093685488989 ) ) ;
#108939=ORIENTED_EDGE ( 'NONE', *, *, #105431, .T. ) ;
#108940=VECTOR ( 'NONE', #98154, 1000.000000000000000 ) ;
#108941=PLANE ( 'NONE',  #92664 ) ;
#108942=CONICAL_SURFACE ( 'NONE', #52535, 0.1000000000000002554, 0.003490658503988666988 ) ;
#108943=CARTESIAN_POINT ( 'NONE',  ( 9.549999999999915445, 12.50000000000000000, -2.230156782645139391 ) ) ;
#108944=ORIENTED_EDGE ( 'NONE', *, *, #79004, .F. ) ;
#108945=AXIS2_PLACEMENT_3D ( 'NONE', #99077, #9408, #46751 ) ;
#108946=CARTESIAN_POINT ( 'NONE',  ( -2.100000000000034284, 2.500000000000000000, -4.330127018922201643 ) ) ;
#108947=DIRECTION ( 'NONE',  ( -4.274815082592931898E-19, -0.9999939076577903929, -0.003490651415223739937 ) ) ;
#108948=EDGE_LOOP ( 'NONE', ( #29281, #100210 ) ) ;
#108949=VERTEX_POINT ( 'NONE', #8953 ) ;
#108950=ORIENTED_EDGE ( 'NONE', *, *, #56283, .F. ) ;
#108951=LINE ( 'NONE', #19289, #23233 ) ;
#108952=CARTESIAN_POINT ( 'NONE',  ( 2.099999999999947686, 2.500000000000000000, 5.022947341949748790 ) ) ;
#108953=CARTESIAN_POINT ( 'NONE',  ( -11.69999999999999574, 12.50000000000000000, 4.265033745738159077 ) ) ;
#108954=FACE_BOUND ( 'NONE', #108182, .T. ) ;
#108955=ORIENTED_EDGE ( 'NONE', *, *, #118379, .T. ) ;
#108956=DIRECTION ( 'NONE',  ( -0.000000000000000000, -1.000000000000000000, -0.000000000000000000 ) ) ;
#108957=DIRECTION ( 'NONE',  ( -0.000000000000000000, 1.000000000000000000, -0.000000000000000000 ) ) ;
#108958=ORIENTED_EDGE ( 'NONE', *, *, #18225, .T. ) ;
#108959=CARTESIAN_POINT ( 'NONE',  ( 2.099999999999949463, 12.50000000000000000, -3.572213422710612374 ) ) ;
#108960=CARTESIAN_POINT ( 'NONE',  ( -8.950000000000009948, 2.500000000000000000, -1.818653347947326138 ) ) ;
#108961=CARTESIAN_POINT ( 'NONE',  ( 7.899999999999924860, 2.500000000000000000, -4.430127018922202176 ) ) ;
#108962=ADVANCED_FACE ( 'NONE', ( #30570 ), #34172, .T. ) ;
#108963=CARTESIAN_POINT ( 'NONE',  ( 7.049999999999926992, 2.500000000000000000, 2.165063509461097713 ) ) ;
#108964=DIRECTION ( 'NONE',  ( -0.000000000000000000, 1.000000000000000000, -0.000000000000000000 ) ) ;
#108965=ADVANCED_FACE ( 'NONE', ( #32507 ), #50204, .T. ) ;
#108966=DIRECTION ( 'NONE',  ( 0.000000000000000000, 0.000000000000000000, 1.000000000000000000 ) ) ;
#108967=DIRECTION ( 'NONE',  ( -0.000000000000000000, 1.000000000000000000, -0.000000000000000000 ) ) ;
#108968=EDGE_CURVE ( 'NONE', #37478, #25981, #107315, .T. ) ;
#108969=CIRCLE ( 'NONE', #10758, 0.06509327318403745899 ) ;
#108970=EDGE_LOOP ( 'NONE', ( #107958, #24516 ) ) ;
#108971=ORIENTED_EDGE ( 'NONE', *, *, #45603, .T. ) ;
#108972=ORIENTED_EDGE ( 'NONE', *, *, #113563, .T. ) ;
#108973=ORIENTED_EDGE ( 'NONE', *, *, #9112, .F. ) ;
#108974=EDGE_LOOP ( 'NONE', ( #18298, #91067 ) ) ;
#108975=CARTESIAN_POINT ( 'NONE',  ( -14.34999999999998543, 12.50000000000000000, 2.576566944158914740 ) ) ;
#108976=EDGE_CURVE ( 'NONE', #128150, #108123, #124038, .T. ) ;
#108977=CARTESIAN_POINT ( 'NONE',  ( 1.649999999999949729, 12.50000000000000000, 7.253104124594885960 ) ) ;
#108978=ORIENTED_EDGE ( 'NONE', *, *, #116178, .T. ) ;
#108979=ADVANCED_FACE ( 'NONE', ( #70469 ), #34271, .T. ) ;
#108980=FACE_BOUND ( 'NONE', #56383, .T. ) ;
#108981=CIRCLE ( 'NONE', #2361, 0.09999999999999982514 ) ;
#108982=FACE_OUTER_BOUND ( 'NONE', #13629, .T. ) ;
#108983=EDGE_CURVE ( 'NONE', #33136, #103573, #31207, .T. ) ;
#108984=AXIS2_PLACEMENT_3D ( 'NONE', #47743, #90215, #127586 ) ;
#108985=ADVANCED_FACE ( 'NONE', ( #22031 ), #89465, .T. ) ;
#108986=ADVANCED_FACE ( 'NONE', ( #61302 ), #55184, .T. ) ;
#108987=DIRECTION ( 'NONE',  ( -0.000000000000000000, -1.000000000000000000, -0.000000000000000000 ) ) ;
#108988=LINE ( 'NONE', #19993, #30375 ) ;
#108989=CARTESIAN_POINT ( 'NONE',  ( -8.550000000000007816, 12.50000000000000000, 6.083687093685482772 ) ) ;
#108990=CARTESIAN_POINT ( 'NONE',  ( 5.599999999999933031, 2.500000000000000000, 0.3464101615137735735 ) ) ;
#108991=DIRECTION ( 'NONE',  ( 0.000000000000000000, 1.000000000000000000, 0.000000000000000000 ) ) ;
#108992=ORIENTED_EDGE ( 'NONE', *, *, #3647, .T. ) ;
#108993=EDGE_CURVE ( 'NONE', #38652, #97177, #40380, .T. ) ;
#108994=AXIS2_PLACEMENT_3D ( 'NONE', #95433, #26688, #66603 ) ;
#108995=ORIENTED_EDGE ( 'NONE', *, *, #26685, .F. ) ;
#108997=AXIS2_PLACEMENT_3D ( 'NONE', #44243, #84167, #34452 ) ;
#108998=ORIENTED_EDGE ( 'NONE', *, *, #83900, .F. ) ;
#108999=ORIENTED_EDGE ( 'NONE', *, *, #9053, .T. ) ;
#109000=CONICAL_SURFACE ( 'NONE', #52583, 0.1000000000000002554, 0.003490658503988666988 ) ;
#109001=DIRECTION ( 'NONE',  ( 0.000000000000000000, -0.000000000000000000, 1.000000000000000000 ) ) ;
#109002=CARTESIAN_POINT ( 'NONE',  ( -15.79999999999998117, 2.500000000000000000, 0.000000000000000000 ) ) ;
#109003=VERTEX_POINT ( 'NONE', #80303 ) ;
#109004=DIRECTION ( 'NONE',  ( -0.000000000000000000, 1.000000000000000000, -0.000000000000000000 ) ) ;
#109005=AXIS2_PLACEMENT_3D ( 'NONE', #50083, #88693, #89969 ) ;
#109006=CARTESIAN_POINT ( 'NONE',  ( 0.8499999999999550138, 2.500000000000000000, -5.802370205355749988 ) ) ;
#109007=DIRECTION ( 'NONE',  ( 0.000000000000000000, 0.000000000000000000, -1.000000000000000000 ) ) ;
#109008=AXIS2_PLACEMENT_3D ( 'NONE', #126551, #36884, #25762 ) ;
#109009=CIRCLE ( 'NONE', #90227, 0.06509327318403745899 ) ;
#109011=DIRECTION ( 'NONE',  ( 0.000000000000000000, 0.000000000000000000, -1.000000000000000000 ) ) ;
#109012=CARTESIAN_POINT ( 'NONE',  ( -8.750000000000012434, 2.500000000000000000, -5.702370205355745014 ) ) ;
#109013=CARTESIAN_POINT ( 'NONE',  ( 7.499999999999960032, 2.500000000000000000, -2.276824562219559311E-15 ) ) ;
#109014=ORIENTED_EDGE ( 'NONE', *, *, #64408, .T. ) ;
#109015=CARTESIAN_POINT ( 'NONE',  ( 2.099999999999948574, 2.500000000000000000, 4.330127018922196314 ) ) ;
#109016=ORIENTED_EDGE ( 'NONE', *, *, #90137, .F. ) ;
#109017=EDGE_LOOP ( 'NONE', ( #96043, #36433, #55990, #69913 ) ) ;
#109018=DIRECTION ( 'NONE',  ( 0.000000000000000000, 0.000000000000000000, -1.000000000000000000 ) ) ;
#109019=DIRECTION ( 'NONE',  ( 0.000000000000000000, 0.000000000000000000, -1.000000000000000000 ) ) ;
#109020=FACE_OUTER_BOUND ( 'NONE', #45667, .T. ) ;
#109021=EDGE_LOOP ( 'NONE', ( #38966, #74591 ) ) ;
#109022=EDGE_LOOP ( 'NONE', ( #93216, #124994, #43322, #16810 ) ) ;
#109025=CARTESIAN_POINT ( 'NONE',  ( -1.450000000000035927, 2.500000000000000000, -1.718653347947326049 ) ) ;
#109026=AXIS2_PLACEMENT_3D ( 'NONE', #119593, #69868, #101253 ) ;
#109028=ORIENTED_EDGE ( 'NONE', *, *, #62027, .T. ) ;
#109030=CIRCLE ( 'NONE', #86043, 0.06509327318403745899 ) ;
#109032=ORIENTED_EDGE ( 'NONE', *, *, #120950, .T. ) ;
#109033=CARTESIAN_POINT ( 'NONE',  ( -10.85000000000000142, 12.50000000000000000, 6.430097255199259010 ) ) ;
#109034=ORIENTED_EDGE ( 'NONE', *, *, #40367, .F. ) ;
#109035=DIRECTION ( 'NONE',  ( -0.000000000000000000, -1.000000000000000000, -0.000000000000000000 ) ) ;
#109036=CIRCLE ( 'NONE', #52615, 0.09999999999999982514 ) ;
#109037=DIRECTION ( 'NONE',  ( -4.274815082592931898E-19, -0.9999939076577903929, -0.003490651415223739937 ) ) ;
#109039=EDGE_CURVE ( 'NONE', #5490, #3622, #82388, .T. ) ;
#109040=LINE ( 'NONE', #129379, #25012 ) ;
#109042=AXIS2_PLACEMENT_3D ( 'NONE', #61348, #101265, #11595 ) ;
#109043=LINE ( 'NONE', #99263, #7033 ) ;
#109044=ORIENTED_EDGE ( 'NONE', *, *, #205, .T. ) ;
#109045=ORIENTED_EDGE ( 'NONE', *, *, #95557, .F. ) ;
#109046=DIRECTION ( 'NONE',  ( -4.274815082592931898E-19, -0.9999939076577903929, -0.003490651415223739937 ) ) ;
#109047=DIRECTION ( 'NONE',  ( -0.000000000000000000, 1.000000000000000000, -0.000000000000000000 ) ) ;
#109048=CARTESIAN_POINT ( 'NONE',  ( -11.84999999999999787, 12.50000000000000000, -2.446380397790836270 ) ) ;
#109049=CARTESIAN_POINT ( 'NONE',  ( 7.699999999999922018, 2.500000000000000000, 0.3464101615137735735 ) ) ;
#109050=CARTESIAN_POINT ( 'NONE',  ( 13.54999999999989768, 12.50000000000000000, -2.446380397790840266 ) ) ;
#109051=DIRECTION ( 'NONE',  ( 0.000000000000000000, -0.000000000000000000, 1.000000000000000000 ) ) ;
#109052=PLANE ( 'NONE',  #36365 ) ;
#109053=DIRECTION ( 'NONE',  ( 0.000000000000000000, 1.000000000000000000, 0.000000000000000000 ) ) ;
#109054=CARTESIAN_POINT ( 'NONE',  ( 7.899999999999924860, 12.50000000000000000, -5.022947341949754119 ) ) ;
#109055=CIRCLE ( 'NONE', #127954, 0.1000000000000002554 ) ;
#109056=AXIS2_PLACEMENT_3D ( 'NONE', #97640, #80589, #108099 ) ;
#109057=EDGE_CURVE ( 'NONE', #68357, #126539, #10264, .T. ) ;
#109058=VERTEX_POINT ( 'NONE', #41679 ) ;
#109059=DIRECTION ( 'NONE',  ( -4.274815082592931898E-19, -0.9999939076577903929, -0.003490651415223739937 ) ) ;
#109060=CARTESIAN_POINT ( 'NONE',  ( -7.500000000000001776, 2.500000000000000000, -9.999999999999998224 ) ) ;
#109061=DIRECTION ( 'NONE',  ( 0.000000000000000000, -0.9999939076577903929, 0.003490651415223739937 ) ) ;
#109062=DIRECTION ( 'NONE',  ( 0.000000000000000000, -0.000000000000000000, 1.000000000000000000 ) ) ;
#109063=CARTESIAN_POINT ( 'NONE',  ( -9.600000000000006750, 2.500000000000000000, 0.6928203230275494784 ) ) ;
#109064=CONICAL_SURFACE ( 'NONE', #40149, 0.1000000000000000472, 0.003490658503988666988 ) ;
#109065=EDGE_CURVE ( 'NONE', #38979, #87148, #72414, .T. ) ;
#109066=CIRCLE ( 'NONE', #40150, 0.09999999999999982514 ) ;
#109067=ORIENTED_EDGE ( 'NONE', *, *, #111124, .F. ) ;
#109068=CARTESIAN_POINT ( 'NONE',  ( -8.350000000000012079, 2.500000000000000000, -1.372243186433550033 ) ) ;
#109069=AXIS2_PLACEMENT_3D ( 'NONE', #78671, #87811, #28924 ) ;
#109070=AXIS2_PLACEMENT_3D ( 'NONE', #33123, #73025, #112953 ) ;
#109071=VECTOR ( 'NONE', #13218, 1000.000000000000000 ) ;
#109072=DIRECTION ( 'NONE',  ( 0.000000000000000000, 0.000000000000000000, -1.000000000000000000 ) ) ;
#109073=DIRECTION ( 'NONE',  ( 0.000000000000000000, 0.000000000000000000, -1.000000000000000000 ) ) ;
#109074=ORIENTED_EDGE ( 'NONE', *, *, #3459, .F. ) ;
#109075=EDGE_CURVE ( 'NONE', #47875, #29014, #15452, .T. ) ;
#109076=EDGE_CURVE ( 'NONE', #1255, #123959, #29906, .T. ) ;
#109077=EDGE_CURVE ( 'NONE', #32548, #124869, #25943, .T. ) ;
#109078=EDGE_CURVE ( 'NONE', #37781, #14798, #122164, .T. ) ;
#109079=EDGE_CURVE ( 'NONE', #122539, #22326, #12172, .T. ) ;
#109080=VECTOR ( 'NONE', #16683, 1000.000000000000000 ) ;
#109081=ORIENTED_EDGE ( 'NONE', *, *, #34539, .F. ) ;
#109082=DIRECTION ( 'NONE',  ( 0.000000000000000000, 1.000000000000000000, 0.000000000000000000 ) ) ;
#109083=VERTEX_POINT ( 'NONE', #35074 ) ;
#109084=ORIENTED_EDGE ( 'NONE', *, *, #89057, .F. ) ;
#109085=VECTOR ( 'NONE', #35586, 1000.000000000000000 ) ;
#109086=ORIENTED_EDGE ( 'NONE', *, *, #27403, .F. ) ;
#109087=VECTOR ( 'NONE', #123203, 1000.000000000000000 ) ;
#109088=CARTESIAN_POINT ( 'NONE',  ( -6.650000000000014566, 2.500000000000000000, 2.165063509461097713 ) ) ;
#109089=EDGE_CURVE ( 'NONE', #43890, #51917, #88630, .T. ) ;
#109090=CIRCLE ( 'NONE', #42312, 0.06509327318403743123 ) ;
#109091=CARTESIAN_POINT ( 'NONE',  ( 19.61395058415646986, 2.556813634648396505, -4.305699210822436562 ) ) ;
#109092=DIRECTION ( 'NONE',  ( 0.000000000000000000, 0.000000000000000000, 1.000000000000000000 ) ) ;
#109093=ADVANCED_FACE ( 'NONE', ( #13468 ), #23796, .T. ) ;
#109094=CARTESIAN_POINT ( 'NONE',  ( 16.32066102237061500, 2.500000000000000000, -4.877377760480841040 ) ) ;
#109095=ADVANCED_FACE ( 'NONE', ( #74980 ), #9205, .T. ) ;
#109096=ORIENTED_EDGE ( 'NONE', *, *, #6395, .F. ) ;
#109097=PLANE ( 'NONE',  #44070 ) ;
#109098=VERTEX_POINT ( 'NONE', #65133 ) ;
#109099=DIRECTION ( 'NONE',  ( 0.000000000000000000, 0.000000000000000000, -1.000000000000000000 ) ) ;
#109100=CARTESIAN_POINT ( 'NONE',  ( 19.21290572970781696, 2.587129408759358373, 2.394140119531668720 ) ) ;
#109101=DIRECTION ( 'NONE',  ( 0.000000000000000000, 0.000000000000000000, 1.000000000000000000 ) ) ;
#109102=DIRECTION ( 'NONE',  ( 0.000000000000000000, 0.000000000000000000, 1.000000000000000000 ) ) ;
#109103=VERTEX_POINT ( 'NONE', #123426 ) ;
#109104=ORIENTED_EDGE ( 'NONE', *, *, #97909, .T. ) ;
#109105=EDGE_LOOP ( 'NONE', ( #121610, #33542 ) ) ;
#109106=EDGE_LOOP ( 'NONE', ( #43093, #82377 ) ) ;
#109107=EDGE_LOOP ( 'NONE', ( #78803, #88801, #120665, #86474 ) ) ;
#109108=DIRECTION ( 'NONE',  ( 0.000000000000000000, 0.000000000000000000, 1.000000000000000000 ) ) ;
#109109=DIRECTION ( 'NONE',  ( 0.000000000000000000, 0.000000000000000000, 1.000000000000000000 ) ) ;
#109110=DIRECTION ( 'NONE',  ( 0.000000000000000000, -0.000000000000000000, 1.000000000000000000 ) ) ;
#109111=FACE_BOUND ( 'NONE', #90642, .T. ) ;
#109112=CARTESIAN_POINT ( 'NONE',  ( -8.350000000000012079, 2.500000000000000000, -2.757883832488654097 ) ) ;
#109113=LINE ( 'NONE', #89498, #65153 ) ;
#109114=CARTESIAN_POINT ( 'NONE',  ( 7.949999999999922018, 2.500000000000000000, -2.065063509461102065 ) ) ;
#109115=LINE ( 'NONE', #1748, #110650 ) ;
#109116=AXIS2_PLACEMENT_3D ( 'NONE', #107037, #67092, #47497 ) ;
#109117=AXIS2_PLACEMENT_3D ( 'NONE', #30259, #79349, #29586 ) ;
#109118=CARTESIAN_POINT ( 'NONE',  ( 8.749999999999957367, 2.500000000000000000, 2.165063509461097713 ) ) ;
#109119=AXIS2_PLACEMENT_3D ( 'NONE', #64145, #83788, #43887 ) ;
#109120=DIRECTION ( 'NONE',  ( 0.000000000000000000, -0.000000000000000000, 1.000000000000000000 ) ) ;
#109121=DIRECTION ( 'NONE',  ( 0.000000000000000000, 0.000000000000000000, -1.000000000000000000 ) ) ;
#109122=EDGE_CURVE ( 'NONE', #47582, #37369, #115814, .T. ) ;
#109123=AXIS2_PLACEMENT_3D ( 'NONE', #20362, #31473, #40670 ) ;
#109124=CIRCLE ( 'NONE', #33936, 0.1000000000000002554 ) ;
#109125=DIRECTION ( 'NONE',  ( 0.000000000000000000, 1.000000000000000000, 0.000000000000000000 ) ) ;
#109126=EDGE_CURVE ( 'NONE', #16861, #69482, #59409, .T. ) ;
#109127=AXIS2_PLACEMENT_3D ( 'NONE', #113215, #13069, #53028 ) ;
#109128=ORIENTED_EDGE ( 'NONE', *, *, #128060, .T. ) ;
#109129=ORIENTED_EDGE ( 'NONE', *, *, #20602, .T. ) ;
#109130=ORIENTED_EDGE ( 'NONE', *, *, #85142, .F. ) ;
#109131=ORIENTED_EDGE ( 'NONE', *, *, #40631, .F. ) ;
#109132=AXIS2_PLACEMENT_3D ( 'NONE', #76193, #123989, #15956 ) ;
#109133=DIRECTION ( 'NONE',  ( -0.000000000000000000, 1.000000000000000000, -0.000000000000000000 ) ) ;
#109134=VECTOR ( 'NONE', #44731, 1000.000000000000000 ) ;
#109135=DIRECTION ( 'NONE',  ( -0.000000000000000000, -1.000000000000000000, -0.000000000000000000 ) ) ;
#109136=ADVANCED_FACE ( 'NONE', ( #95271 ), #83524, .T. ) ;
#109137=FACE_BOUND ( 'NONE', #41178, .T. ) ;
#109138=CIRCLE ( 'NONE', #63192, 0.06509327318403745899 ) ;
#109139=DIRECTION ( 'NONE',  ( 0.000000000000000000, 1.000000000000000000, 0.000000000000000000 ) ) ;
#109140=ADVANCED_FACE ( 'NONE', ( #84137 ), #73964, .T. ) ;
#109142=EDGE_LOOP ( 'NONE', ( #8103, #58969, #113927, #46662 ) ) ;
#109143=CARTESIAN_POINT ( 'NONE',  ( 12.89999999999989733, 2.500000000000000000, -0.1000000000000023925 ) ) ;
#109144=CARTESIAN_POINT ( 'NONE',  ( -4.600000000000024514, 12.50000000000000000, 3.637306695894644726 ) ) ;
#109145=DIRECTION ( 'NONE',  ( 0.000000000000000000, 1.000000000000000000, 0.000000000000000000 ) ) ;
#109146=PLANE ( 'NONE',  #87678 ) ;
#109147=CARTESIAN_POINT ( 'NONE',  ( 4.599999999999936584, 12.50000000000000000, 4.330127018922196314 ) ) ;
#109148=ORIENTED_EDGE ( 'NONE', *, *, #34224, .F. ) ;
#109149=CARTESIAN_POINT ( 'NONE',  ( 0.8499999999999545697, 2.500000000000000000, -1.372243186433550033 ) ) ;
#109150=ADVANCED_FACE ( 'NONE', ( #105064 ), #126291, .T. ) ;
#109151=EDGE_LOOP ( 'NONE', ( #28702, #105319, #59297, #82492 ) ) ;
#109152=ORIENTED_EDGE ( 'NONE', *, *, #111733, .T. ) ;
#109153=DIRECTION ( 'NONE',  ( 0.000000000000000000, 0.000000000000000000, 1.000000000000000000 ) ) ;
#109154=DIRECTION ( 'NONE',  ( 0.000000000000000000, -0.9999939076577903929, 0.003490651415223739937 ) ) ;
#109155=EDGE_LOOP ( 'NONE', ( #75547, #10053 ) ) ;
#109156=AXIS2_PLACEMENT_3D ( 'NONE', #108919, #89934, #91235 ) ;
#109157=DIRECTION ( 'NONE',  ( -4.274815082592931898E-19, -0.9999939076577903929, -0.003490651415223739937 ) ) ;
#109158=CARTESIAN_POINT ( 'NONE',  ( -4.200000000000025935, 2.500000000000000000, -2.385244779468109755E-15 ) ) ;
#109159=VERTEX_POINT ( 'NONE', #125369 ) ;
#109160=PLANE ( 'NONE',  #61979 ) ;
#109161=EDGE_LOOP ( 'NONE', ( #57321, #60322, #65798, #106960 ) ) ;
#109162=CARTESIAN_POINT ( 'NONE',  ( 11.24999999999994493, 2.500000000000000000, 6.395190528383296602 ) ) ;
#109163=EDGE_CURVE ( 'NONE', #27375, #118968, #30063, .T. ) ;
#109165=EDGE_LOOP ( 'NONE', ( #842, #111987, #64378, #54406 ) ) ;
#109167=FACE_BOUND ( 'NONE', #36708, .T. ) ;
#109168=AXIS2_PLACEMENT_3D ( 'NONE', #52504, #121897, #74735 ) ;
#109169=EDGE_LOOP ( 'NONE', ( #112335, #106921 ) ) ;
#109170=CIRCLE ( 'NONE', #69467, 0.06509327318403745899 ) ;
#109171=CARTESIAN_POINT ( 'NONE',  ( -8.950000000000006395, 2.500000000000000000, 6.941600689897073018 ) ) ;
#109172=ORIENTED_EDGE ( 'NONE', *, *, #53121, .F. ) ;
#109173=DIRECTION ( 'NONE',  ( -0.000000000000000000, 1.000000000000000000, -0.000000000000000000 ) ) ;
#109174=CARTESIAN_POINT ( 'NONE',  ( -8.150000000000014566, 12.50000000000000000, -6.776507416713036136 ) ) ;
#109175=FACE_OUTER_BOUND ( 'NONE', #8208, .T. ) ;
#109176=DIRECTION ( 'NONE',  ( 0.000000000000000000, 0.000000000000000000, 1.000000000000000000 ) ) ;
#109177=CARTESIAN_POINT ( 'NONE',  ( 17.28960762337857915, 1.567482926518815267, -5.035524966326118346 ) ) ;
#109178=AXIS2_PLACEMENT_3D ( 'NONE', #48113, #119405, #29754 ) ;
#109179=ORIENTED_EDGE ( 'NONE', *, *, #68764, .T. ) ;
#109180=ORIENTED_EDGE ( 'NONE', *, *, #79556, .F. ) ;
#109181=VECTOR ( 'NONE', #51844, 1000.000000000000000 ) ;
#109182=EDGE_LOOP ( 'NONE', ( #127545, #78689 ) ) ;
#109183=CARTESIAN_POINT ( 'NONE',  ( -3.950000000000026379, 2.500000000000000000, 6.841600689897072485 ) ) ;
#109184=EDGE_CURVE ( 'NONE', #104949, #66592, #73676, .T. ) ;
#109185=DIRECTION ( 'NONE',  ( 0.000000000000000000, -0.9999939076577903929, 0.003490651415223739937 ) ) ;
#109186=AXIS2_PLACEMENT_3D ( 'NONE', #39218, #49026, #109200 ) ;
#109187=AXIS2_PLACEMENT_3D ( 'NONE', #17764, #48528, #37434 ) ;
#109188=AXIS2_PLACEMENT_3D ( 'NONE', #63637, #32260, #2767 ) ;
#109189=CARTESIAN_POINT ( 'NONE',  ( 15.39999999999989200, 2.500000000000000000, -0.5928203230275542746 ) ) ;
#109190=EDGE_LOOP ( 'NONE', ( #88928, #23015 ) ) ;
#109191=ORIENTED_EDGE ( 'NONE', *, *, #35425, .F. ) ;
#109192=ORIENTED_EDGE ( 'NONE', *, *, #119476, .F. ) ;
#109193=CARTESIAN_POINT ( 'NONE',  ( -1.250000000000001554, 2.500000000000000000, 2.265063509461097357 ) ) ;
#109194=CONICAL_SURFACE ( 'NONE', #46498, 0.09999999999999982514, 0.003490658503988666988 ) ;
#109195=CARTESIAN_POINT ( 'NONE',  ( 1.049999999999953637, 12.50000000000000000, -1.753560074763288679 ) ) ;
#109197=CARTESIAN_POINT ( 'NONE',  ( -2.700000000000029932, 12.50000000000000000, -0.2813168883297408329 ) ) ;
#109198=CIRCLE ( 'NONE', #38215, 0.06509327318403745899 ) ;
#109199=CARTESIAN_POINT ( 'NONE',  ( -1.050000000000037792, 2.500000000000000000, 6.148780366869520009 ) ) ;
#109200=DIRECTION ( 'NONE',  ( 0.000000000000000000, -0.000000000000000000, 1.000000000000000000 ) ) ;
#109203=ADVANCED_FACE ( 'NONE', ( #23952 ), #115523, .T. ) ;
#109204=FACE_OUTER_BOUND ( 'NONE', #22951, .T. ) ;
#109205=ORIENTED_EDGE ( 'NONE', *, *, #69836, .T. ) ;
#109206=ORIENTED_EDGE ( 'NONE', *, *, #96126, .F. ) ;
#109207=CARTESIAN_POINT ( 'NONE',  ( -0.4500000000000397571, 2.500000000000000000, -2.265063509461101798 ) ) ;
#109208=DIRECTION ( 'NONE',  ( 0.000000000000000000, 0.000000000000000000, -1.000000000000000000 ) ) ;
#109209=EDGE_LOOP ( 'NONE', ( #119798, #76985 ) ) ;
#109210=EDGE_LOOP ( 'NONE', ( #118414, #20243 ) ) ;
#109211=VECTOR ( 'NONE', #69468, 1000.000000000000000 ) ;
#109213=DIRECTION ( 'NONE',  ( 1.000000000000000000, 0.000000000000000000, 0.000000000000000000 ) ) ;
#109214=CARTESIAN_POINT ( 'NONE',  ( 3.949999999999938893, 2.500000000000000000, 6.148780366869520009 ) ) ;
#109215=DIRECTION ( 'NONE',  ( 0.000000000000000000, 0.000000000000000000, -1.000000000000000000 ) ) ;
#109216=CARTESIAN_POINT ( 'NONE',  ( -6.050000000000022027, 12.50000000000000000, -6.213873640053564351 ) ) ;
#109218=CARTESIAN_POINT ( 'NONE',  ( 1.249999999999952038, 12.50000000000000000, 2.792790559304612064 ) ) ;
#109219=FACE_OUTER_BOUND ( 'NONE', #114735, .T. ) ;
#109220=CIRCLE ( 'NONE', #42338, 0.06509327318403745899 ) ;
#109221=VECTOR ( 'NONE', #117739, 1000.000000000000000 ) ;
#109222=CARTESIAN_POINT ( 'NONE',  ( 5.399999999999935518, 2.500000000000000000, -4.230127018922201998 ) ) ;
#109223=VECTOR ( 'NONE', #127585, 1000.000000000000000 ) ;
#109224=ORIENTED_EDGE ( 'NONE', *, *, #72266, .T. ) ;
#109225=VECTOR ( 'NONE', #19585, 1000.000000000000000 ) ;
#109226=EDGE_CURVE ( 'NONE', #116825, #15903, #124073, .T. ) ;
#109227=ORIENTED_EDGE ( 'NONE', *, *, #16173, .T. ) ;
#109228=AXIS2_PLACEMENT_3D ( 'NONE', #76520, #73442, #125594 ) ;
#109229=AXIS2_PLACEMENT_3D ( 'NONE', #96158, #34693, #75873 ) ;
#109230=EDGE_LOOP ( 'NONE', ( #23345, #86225 ) ) ;
#109231=ORIENTED_EDGE ( 'NONE', *, *, #52214, .F. ) ;
#109232=DIRECTION ( 'NONE',  ( 0.000000000000000000, 1.000000000000000000, 0.000000000000000000 ) ) ;
#109233=DIRECTION ( 'NONE',  ( 0.000000000000000000, 1.000000000000000000, 0.000000000000000000 ) ) ;
#109234=CIRCLE ( 'NONE', #113452, 0.09999999999999999167 ) ;
#109235=ADVANCED_FACE ( 'NONE', ( #44220 ), #13306, .T. ) ;
#109236=EDGE_LOOP ( 'NONE', ( #76146, #54023, #85267, #29550 ) ) ;
#109237=DIRECTION ( 'NONE',  ( 0.000000000000000000, 1.000000000000000000, 0.000000000000000000 ) ) ;
#109238=CARTESIAN_POINT ( 'NONE',  ( 3.549999999999944755, 2.500000000000000000, -2.511473670974877948 ) ) ;
#109239=DIRECTION ( 'NONE',  ( 0.000000000000000000, 1.000000000000000000, 0.000000000000000000 ) ) ;
#109240=LINE ( 'NONE', #30725, #22440 ) ;
#109241=ORIENTED_EDGE ( 'NONE', *, *, #26699, .F. ) ;
#109242=ADVANCED_FACE ( 'NONE', ( #74333 ), #105358, .T. ) ;
#109243=ADVANCED_FACE ( 'NONE', ( #14108 ), #124128, .T. ) ;
#109244=EDGE_CURVE ( 'NONE', #104766, #41779, #63507, .T. ) ;
#109245=CARTESIAN_POINT ( 'NONE',  ( 2.500000000000002220, -1.500000000000000000, -9.999999999999998224 ) ) ;
#109246=EDGE_CURVE ( 'NONE', #102257, #90767, #55970, .T. ) ;
#109247=AXIS2_PLACEMENT_3D ( 'NONE', #104915, #103661, #83994 ) ;
#109248=FACE_OUTER_BOUND ( 'NONE', #66051, .T. ) ;
#109249=ORIENTED_EDGE ( 'NONE', *, *, #12052, .T. ) ;
#109250=EDGE_CURVE ( 'NONE', #11624, #9428, #108299, .T. ) ;
#109251=ORIENTED_EDGE ( 'NONE', *, *, #120447, .T. ) ;
#109252=ADVANCED_FACE ( 'NONE', ( #127311 ), #44730, .T. ) ;
#109253=VERTEX_POINT ( 'NONE', #126663 ) ;
#109254=VERTEX_POINT ( 'NONE', #106997 ) ;
#109255=DIRECTION ( 'NONE',  ( 0.000000000000000000, 1.000000000000000000, 0.000000000000000000 ) ) ;
#109256=EDGE_CURVE ( 'NONE', #96511, #109502, #101158, .T. ) ;
#109257=ADVANCED_FACE ( 'NONE', ( #67058 ), #13401, .T. ) ;
#109258=CARTESIAN_POINT ( 'NONE',  ( 7.899999999999924860, 2.500000000000000000, -5.022947341949754119 ) ) ;
#109259=AXIS2_PLACEMENT_3D ( 'NONE', #84636, #34264, #22516 ) ;
#109260=CARTESIAN_POINT ( 'NONE',  ( -0.8500000000000386136, 12.50000000000000000, 1.472243186433545459 ) ) ;
#109261=CONICAL_SURFACE ( 'NONE', #109358, 0.1000000000000000472, 0.003490658503988666988 ) ;
#109262=EDGE_CURVE ( 'NONE', #58840, #73617, #32320, .T. ) ;
#109263=CIRCLE ( 'NONE', #90468, 0.06509327318403745899 ) ;
#109264=EDGE_CURVE ( 'NONE', #73752, #63793, #97198, .T. ) ;
#109265=ORIENTED_EDGE ( 'NONE', *, *, #55626, .T. ) ;
#109266=CARTESIAN_POINT ( 'NONE',  ( 2.499999999999947153, 12.50000000000000000, -3.637306695894650055 ) ) ;
#109267=DIRECTION ( 'NONE',  ( 0.000000000000000000, 1.000000000000000000, 0.000000000000000000 ) ) ;
#109268=DIRECTION ( 'NONE',  ( 0.000000000000000000, 0.000000000000000000, -1.000000000000000000 ) ) ;
#109270=AXIS2_PLACEMENT_3D ( 'NONE', #57628, #75317, #36052 ) ;
#109271=EDGE_CURVE ( 'NONE', #126334, #105882, #53230, .T. ) ;
#109272=CONICAL_SURFACE ( 'NONE', #67486, 0.1000000000000002554, 0.003490658503988666988 ) ;
#109273=AXIS2_PLACEMENT_3D ( 'NONE', #47211, #5970, #87755 ) ;
#109274=ORIENTED_EDGE ( 'NONE', *, *, #8890, .F. ) ;
#109275=DIRECTION ( 'NONE',  ( 0.000000000000000000, -0.000000000000000000, 1.000000000000000000 ) ) ;
#109276=CIRCLE ( 'NONE', #115620, 0.1000000000000002554 ) ;
#109277=ORIENTED_EDGE ( 'NONE', *, *, #49453, .T. ) ;
#109278=ORIENTED_EDGE ( 'NONE', *, *, #35929, .T. ) ;
#109279=CARTESIAN_POINT ( 'NONE',  ( 6.049999999999932321, 12.50000000000000000, 6.776507416713035248 ) ) ;
#109280=DIRECTION ( 'NONE',  ( -0.000000000000000000, 1.000000000000000000, -0.000000000000000000 ) ) ;
#109281=FACE_BOUND ( 'NONE', #40392, .T. ) ;
#109282=FACE_OUTER_BOUND ( 'NONE', #51843, .T. ) ;
#109283=DIRECTION ( 'NONE',  ( 0.000000000000000000, 1.000000000000000000, 0.000000000000000000 ) ) ;
#109284=CIRCLE ( 'NONE', #23506, 0.09999999999999982514 ) ;
#109285=AXIS2_PLACEMENT_3D ( 'NONE', #126378, #66792, #7879 ) ;
#109286=DIRECTION ( 'NONE',  ( 0.000000000000000000, 0.000000000000000000, 1.000000000000000000 ) ) ;
#109287=CIRCLE ( 'NONE', #86286, 0.06509327318403745899 ) ;
#109288=CIRCLE ( 'NONE', #52864, 0.1000000000000002554 ) ;
#109289=ORIENTED_EDGE ( 'NONE', *, *, #127267, .T. ) ;
#109290=FACE_OUTER_BOUND ( 'NONE', #6097, .T. ) ;
#109291=PLANE ( 'NONE',  #40613 ) ;
#109292=CARTESIAN_POINT ( 'NONE',  ( 2.899999999999946620, 2.500000000000000000, 0.7928203230275495672 ) ) ;
#109293=AXIS2_PLACEMENT_3D ( 'NONE', #20779, #108503, #58770 ) ;
#109294=CARTESIAN_POINT ( 'NONE',  ( -10.60000000000000142, 2.500000000000000000, -0.3464101615137782364 ) ) ;
#109295=ORIENTED_EDGE ( 'NONE', *, *, #16603, .T. ) ;
#109296=FACE_OUTER_BOUND ( 'NONE', #110584, .T. ) ;
#109297=DIRECTION ( 'NONE',  ( -0.000000000000000000, 1.000000000000000000, -0.000000000000000000 ) ) ;
#109298=CIRCLE ( 'NONE', #36158, 0.06509327318403745899 ) ;
#109299=VERTEX_POINT ( 'NONE', #58577 ) ;
#109300=ORIENTED_EDGE ( 'NONE', *, *, #17137, .T. ) ;
#109301=CARTESIAN_POINT ( 'NONE',  ( -11.64999999999999680, 12.50000000000000000, -7.188010851410850499 ) ) ;
#109302=LINE ( 'NONE', #59597, #84068 ) ;
#109303=FACE_BOUND ( 'NONE', #44384, .T. ) ;
#109304=DIRECTION ( 'NONE',  ( -0.000000000000000000, 1.000000000000000000, -0.000000000000000000 ) ) ;
#109305=ADVANCED_FACE ( 'NONE', ( #36363 ), #126376, .T. ) ;
#109306=CARTESIAN_POINT ( 'NONE',  ( -6.250000000000017764, 2.500000000000000000, 2.957883832488649389 ) ) ;
#109307=ADVANCED_FACE ( 'NONE', ( #87363 ), #120031, .T. ) ;
#109308=VECTOR ( 'NONE', #79284, 1000.000000000000000 ) ;
#109309=VERTEX_POINT ( 'NONE', #37646 ) ;
#109310=LINE ( 'NONE', #77909, #94741 ) ;
#109311=AXIS2_PLACEMENT_3D ( 'NONE', #15695, #23599, #84459 ) ;
#109313=ORIENTED_EDGE ( 'NONE', *, *, #85031, .T. ) ;
#109314=CARTESIAN_POINT ( 'NONE',  ( -3.950000000000029932, 2.500000000000000000, -6.148780366869526226 ) ) ;
#109315=DIRECTION ( 'NONE',  ( 0.000000000000000000, 1.000000000000000000, 0.000000000000000000 ) ) ;
#109316=ADVANCED_FACE ( 'NONE', ( #48103 ), #107668, .T. ) ;
#109317=VECTOR ( 'NONE', #17485, 1000.000000000000000 ) ;
#109318=AXIS2_PLACEMENT_3D ( 'NONE', #127040, #9824, #34957 ) ;
#109319=AXIS2_PLACEMENT_3D ( 'NONE', #19515, #110479, #18221 ) ;
#109320=CIRCLE ( 'NONE', #69613, 0.09999999999999982514 ) ;
#109321=DIRECTION ( 'NONE',  ( 0.000000000000000000, 1.000000000000000000, 0.000000000000000000 ) ) ;
#109322=CARTESIAN_POINT ( 'NONE',  ( -7.050000000000016698, 12.50000000000000000, -6.495190528383302464 ) ) ;
#109323=AXIS2_PLACEMENT_3D ( 'NONE', #16938, #78505, #86351 ) ;
#109324=CONICAL_SURFACE ( 'NONE', #75875, 0.1000000000000000472, 0.003490658503988666988 ) ;
#109325=ORIENTED_EDGE ( 'NONE', *, *, #68644, .T. ) ;
#109326=AXIS2_PLACEMENT_3D ( 'NONE', #60496, #100402, #91871 ) ;
#109327=CARTESIAN_POINT ( 'NONE',  ( 7.699999999999925571, 12.50000000000000000, -4.611443907251940644 ) ) ;
#109328=CARTESIAN_POINT ( 'NONE',  ( -11.84999999999999609, 2.500000000000000000, 1.718653347947321386 ) ) ;
#109329=CIRCLE ( 'NONE', #67546, 0.09999999999999982514 ) ;
#109330=CARTESIAN_POINT ( 'NONE',  ( 10.39999999999991509, 2.500000000000000000, -0.6928203230275542523 ) ) ;
#109331=AXIS2_PLACEMENT_3D ( 'NONE', #81052, #73157, #22144 ) ;
#109332=EDGE_LOOP ( 'NONE', ( #126043, #83572 ) ) ;
#109333=EDGE_LOOP ( 'NONE', ( #58450, #114217, #99738, #19871 ) ) ;
#109334=CARTESIAN_POINT ( 'NONE',  ( 17.50982737979238735, 2.500000000000000000, 4.074750942089363726 ) ) ;
#109335=VECTOR ( 'NONE', #29555, 1000.000000000000000 ) ;
#109336=VERTEX_POINT ( 'NONE', #95905 ) ;
#109337=FACE_OUTER_BOUND ( 'NONE', #16054, .T. ) ;
#109338=CARTESIAN_POINT ( 'NONE',  ( 87.50000000000002842, -7.402262750143065340, -1.385127402881715764 ) ) ;
#109339=CARTESIAN_POINT ( 'NONE',  ( -0.6000000000000388356, 12.50000000000000000, 4.676537180435972552 ) ) ;
#109340=EDGE_LOOP ( 'NONE', ( #3236, #41597 ) ) ;
#109341=DIRECTION ( 'NONE',  ( 0.000000000000000000, 0.000000000000000000, 1.000000000000000000 ) ) ;
#109342=FACE_OUTER_BOUND ( 'NONE', #45573, .T. ) ;
#109343=DIRECTION ( 'NONE',  ( -0.000000000000000000, 1.000000000000000000, -0.000000000000000000 ) ) ;
#109345=DIRECTION ( 'NONE',  ( 0.000000000000000000, 1.000000000000000000, 0.000000000000000000 ) ) ;
#109346=CARTESIAN_POINT ( 'NONE',  ( -8.550000000000007816, 12.50000000000000000, 6.148780366869520009 ) ) ;
#109347=CIRCLE ( 'NONE', #50868, 0.06509327318403745899 ) ;
#109348=ORIENTED_EDGE ( 'NONE', *, *, #75144, .F. ) ;
#109349=VERTEX_POINT ( 'NONE', #26526 ) ;
#109350=DIRECTION ( 'NONE',  ( -0.000000000000000000, 1.000000000000000000, -0.000000000000000000 ) ) ;
#109351=ORIENTED_EDGE ( 'NONE', *, *, #29892, .F. ) ;
#109352=CARTESIAN_POINT ( 'NONE',  ( -7.300000000000018474, 2.500000000000000000, 0.3464101615137735735 ) ) ;
#109353=EDGE_LOOP ( 'NONE', ( #82070, #101423 ) ) ;
#109355=VERTEX_POINT ( 'NONE', #88665 ) ;
#109356=PLANE ( 'NONE',  #1925 ) ;
#109357=CIRCLE ( 'NONE', #59206, 0.06509327318403745899 ) ;
#109358=AXIS2_PLACEMENT_3D ( 'NONE', #964, #63105, #40924 ) ;
#109359=DIRECTION ( 'NONE',  ( 0.000000000000000000, 1.000000000000000000, 0.000000000000000000 ) ) ;
#109360=CARTESIAN_POINT ( 'NONE',  ( 1.899999999999949507, 2.500000000000000000, 4.676537180435972552 ) ) ;
#109362=CARTESIAN_POINT ( 'NONE',  ( 13.54999999999990123, 2.500000000000000000, 1.818653347947321475 ) ) ;
#109363=PLANE ( 'NONE',  #104505 ) ;
#109364=DIRECTION ( 'NONE',  ( 0.000000000000000000, 0.000000000000000000, 1.000000000000000000 ) ) ;
#109365=ADVANCED_FACE ( 'NONE', ( #87995 ), #19771, .T. ) ;
#109366=PLANE ( 'NONE',  #16222 ) ;
#109367=CARTESIAN_POINT ( 'NONE',  ( 0.5999999999999621192, 2.500000000000000000, 0.3464101615137758494 ) ) ;
#109368=EDGE_CURVE ( 'NONE', #35141, #117766, #118120, .T. ) ;
#109369=AXIS2_PLACEMENT_3D ( 'NONE', #124280, #47016, #67245 ) ;
#109370=AXIS2_PLACEMENT_3D ( 'NONE', #37116, #98578, #118241 ) ;
#109371=CARTESIAN_POINT ( 'NONE',  ( -0.4500000000000402012, 2.500000000000000000, 2.165063509461097713 ) ) ;
#109372=VERTEX_POINT ( 'NONE', #125997 ) ;
#109373=AXIS2_PLACEMENT_3D ( 'NONE', #102105, #24673, #21610 ) ;
#109374=ORIENTED_EDGE ( 'NONE', *, *, #53901, .T. ) ;
#109375=VECTOR ( 'NONE', #123111, 1000.000000000000000 ) ;
#109376=CARTESIAN_POINT ( 'NONE',  ( 7.699999999999923794, 12.50000000000000000, -3.983716857408426293 ) ) ;
#109377=ORIENTED_EDGE ( 'NONE', *, *, #15312, .F. ) ;
#109378=ADVANCED_FACE ( 'NONE', ( #128624 ), #38960, .T. ) ;
#109379=ORIENTED_EDGE ( 'NONE', *, *, #80297, .F. ) ;
#109380=DIRECTION ( 'NONE',  ( 0.000000000000000000, 0.000000000000000000, -1.000000000000000000 ) ) ;
#109382=CARTESIAN_POINT ( 'NONE',  ( -0.4000000000000396572, 2.500000000000000000, 4.330127018922196314 ) ) ;
#109383=CARTESIAN_POINT ( 'NONE',  ( -10.40000000000000391, 2.500000000000000000, -3.637306695894645614 ) ) ;
#109384=AXIS2_PLACEMENT_3D ( 'NONE', #18597, #119365, #127909 ) ;
#109385=CIRCLE ( 'NONE', #92666, 0.06509327318403745899 ) ;
#109386=CARTESIAN_POINT ( 'NONE',  ( 9.549999999999918998, 12.50000000000000000, -6.495190528383302464 ) ) ;
#109387=ORIENTED_EDGE ( 'NONE', *, *, #7721, .F. ) ;
#109388=ORIENTED_EDGE ( 'NONE', *, *, #85250, .T. ) ;
#109389=CARTESIAN_POINT ( 'NONE',  ( 5.449999999999934452, 2.500000000000000000, 2.165063509461097713 ) ) ;
#109390=ORIENTED_EDGE ( 'NONE', *, *, #124240, .F. ) ;
#109392=EDGE_CURVE ( 'NONE', #111853, #1262, #23894, .T. ) ;
#109393=EDGE_LOOP ( 'NONE', ( #3069, #122954 ) ) ;
#109394=ORIENTED_EDGE ( 'NONE', *, *, #55447, .F. ) ;
#109395=CARTESIAN_POINT ( 'NONE',  ( -6.900000000000015454, 2.500000000000000000, 4.083716857408420609 ) ) ;
#109396=CARTESIAN_POINT ( 'NONE',  ( 12.49999999999990230, 12.50000000000000000, -0.6928203230275541413 ) ) ;
#109397=EDGE_CURVE ( 'NONE', #72434, #18337, #92937, .T. ) ;
#109398=PLANE ( 'NONE',  #19446 ) ;
#109399=CARTESIAN_POINT ( 'NONE',  ( 6.649999999999930189, 2.500000000000000000, 5.802370205355744659 ) ) ;
#109400=DIRECTION ( 'NONE',  ( 0.000000000000000000, 0.000000000000000000, 1.000000000000000000 ) ) ;
#109401=ORIENTED_EDGE ( 'NONE', *, *, #64794, .T. ) ;
#109402=CARTESIAN_POINT ( 'NONE',  ( 1.249999999999952038, 12.50000000000000000, 2.857883832488649301 ) ) ;
#109403=DIRECTION ( 'NONE',  ( -0.000000000000000000, -1.000000000000000000, -0.000000000000000000 ) ) ;
#109404=AXIS2_PLACEMENT_3D ( 'NONE', #13080, #24219, #104063 ) ;
#109405=EDGE_CURVE ( 'NONE', #90044, #117253, #110869, .T. ) ;
#109406=AXIS2_PLACEMENT_3D ( 'NONE', #8240, #67810, #86806 ) ;
#109407=ADVANCED_FACE ( 'NONE', ( #42148 ), #9300, .T. ) ;
#109408=CARTESIAN_POINT ( 'NONE',  ( -15.39999999999998082, 12.50000000000000000, 0.7579135962115892688 ) ) ;
#109409=EDGE_CURVE ( 'NONE', #92182, #21147, #97038, .T. ) ;
#109410=CARTESIAN_POINT ( 'NONE',  ( -13.74999999999995381, 12.50000000000000000, 2.165063509461101265 ) ) ;
#109411=EDGE_CURVE ( 'NONE', #52245, #6156, #51085, .T. ) ;
#109412=CARTESIAN_POINT ( 'NONE',  ( -3.100000000000028955, 12.50000000000000000, 3.918623584224383727 ) ) ;
#109413=ORIENTED_EDGE ( 'NONE', *, *, #5101, .F. ) ;
#109414=AXIS2_PLACEMENT_3D ( 'NONE', #35078, #114895, #63232 ) ;
#109415=CIRCLE ( 'NONE', #96882, 0.1000000000000002554 ) ;
#109416=AXIS2_PLACEMENT_3D ( 'NONE', #38511, #6412, #78438 ) ;
#109417=ORIENTED_EDGE ( 'NONE', *, *, #73201, .T. ) ;
#109419=EDGE_CURVE ( 'NONE', #44266, #74448, #3048, .T. ) ;
#109420=AXIS2_PLACEMENT_3D ( 'NONE', #5399, #95080, #44694 ) ;
#109421=LINE ( 'NONE', #19760, #63368 ) ;
#109422=EDGE_CURVE ( 'NONE', #42047, #101516, #7134, .T. ) ;
#109423=ORIENTED_EDGE ( 'NONE', *, *, #10409, .T. ) ;
#109424=CARTESIAN_POINT ( 'NONE',  ( -4.150000000000025224, 12.50000000000000000, 7.188010851410848723 ) ) ;
#109425=CARTESIAN_POINT ( 'NONE',  ( 8.299999999999922551, 12.50000000000000000, -4.395220292106239768 ) ) ;
#109426=VECTOR ( 'NONE', #63215, 1000.000000000000000 ) ;
#109427=CIRCLE ( 'NONE', #92702, 0.1000000000000002554 ) ;
#109428=EDGE_CURVE ( 'NONE', #88657, #66180, #69666, .T. ) ;
#109429=VECTOR ( 'NONE', #13262, 1000.000000000000000 ) ;
#109430=VERTEX_POINT ( 'NONE', #71601 ) ;
#109431=CARTESIAN_POINT ( 'NONE',  ( 4.999999999999971578, 12.50000000000000000, -2.276824562219559311E-15 ) ) ;
#109432=DIRECTION ( 'NONE',  ( 0.000000000000000000, 0.000000000000000000, 1.000000000000000000 ) ) ;
#109433=ADVANCED_FACE ( 'NONE', ( #111528 ), #31061, .T. ) ;
#109434=DIRECTION ( 'NONE',  ( 0.000000000000000000, 1.000000000000000000, 0.000000000000000000 ) ) ;
#109435=CARTESIAN_POINT ( 'NONE',  ( 4.149999999999939959, 12.50000000000000000, 2.857883832488649301 ) ) ;
#109436=ADVANCED_FACE ( 'NONE', ( #129267 ), #13484, .T. ) ;
#109438=VERTEX_POINT ( 'NONE', #59229 ) ;
#109440=DIRECTION ( 'NONE',  ( 0.000000000000000000, 0.000000000000000000, -1.000000000000000000 ) ) ;
#109441=DIRECTION ( 'NONE',  ( 0.000000000000000000, -0.000000000000000000, 1.000000000000000000 ) ) ;
#109442=CARTESIAN_POINT ( 'NONE',  ( -0.6500000000000394351, 2.500000000000000000, 2.611473670974873151 ) ) ;
#109443=AXIS2_PLACEMENT_3D ( 'NONE', #64207, #101566, #2701 ) ;
#109444=VERTEX_POINT ( 'NONE', #119397 ) ;
#109445=DIRECTION ( 'NONE',  ( 0.000000000000000000, 0.000000000000000000, -1.000000000000000000 ) ) ;
#109446=ORIENTED_EDGE ( 'NONE', *, *, #74986, .F. ) ;
#109447=FACE_OUTER_BOUND ( 'NONE', #51608, .T. ) ;
#109448=CARTESIAN_POINT ( 'NONE',  ( 0.4499999999999552136, 12.50000000000000000, 6.495190528383297135 ) ) ;
#109449=CARTESIAN_POINT ( 'NONE',  ( -12.49999999999999289, 12.50000000000000000, -5.088040615133788691 ) ) ;
#109450=AXIS2_PLACEMENT_3D ( 'NONE', #62115, #22843, #71268 ) ;
#109451=ORIENTED_EDGE ( 'NONE', *, *, #126707, .F. ) ;
#109452=AXIS2_PLACEMENT_3D ( 'NONE', #57154, #57807, #88540 ) ;
#109453=AXIS2_PLACEMENT_3D ( 'NONE', #33779, #63889, #55360 ) ;
#109454=CARTESIAN_POINT ( 'NONE',  ( 5.599999999999931255, 2.500000000000000000, 4.676537180435972552 ) ) ;
#109455=DIRECTION ( 'NONE',  ( 0.000000000000000000, 0.000000000000000000, -1.000000000000000000 ) ) ;
#109456=ORIENTED_EDGE ( 'NONE', *, *, #95935, .T. ) ;
#109457=DIRECTION ( 'NONE',  ( 0.000000000000000000, 0.000000000000000000, -1.000000000000000000 ) ) ;
#109458=AXIS2_PLACEMENT_3D ( 'NONE', #19465, #128815, #80338 ) ;
#109459=ORIENTED_EDGE ( 'NONE', *, *, #44375, .F. ) ;
#109460=VECTOR ( 'NONE', #21322, 1000.000000000000000 ) ;
#109461=CARTESIAN_POINT ( 'NONE',  ( -7.500000000000001776, 1.500000000000000000, 9.000000000000001776 ) ) ;
#109462=AXIS2_PLACEMENT_3D ( 'NONE', #41906, #11778, #74419 ) ;
#109463=EDGE_CURVE ( 'NONE', #11053, #4868, #109656, .T. ) ;
#109464=ORIENTED_EDGE ( 'NONE', *, *, #75560, .F. ) ;
#109465=CARTESIAN_POINT ( 'NONE',  ( 11.44999999999990870, 12.50000000000000000, -1.818653347947326138 ) ) ;
#109466=CARTESIAN_POINT ( 'NONE',  ( -12.49999999999995914, 2.500000000000000000, -0.09999999999999815981 ) ) ;
#109467=EDGE_CURVE ( 'NONE', #118617, #9793, #99784, .T. ) ;
#109468=ORIENTED_EDGE ( 'NONE', *, *, #21342, .T. ) ;
#109469=EDGE_LOOP ( 'NONE', ( #88439, #71717, #18131, #73524 ) ) ;
#109470=CIRCLE ( 'NONE', #59328, 0.06509327318403745899 ) ;
#109471=CARTESIAN_POINT ( 'NONE',  ( -7.100000000000014744, 2.500000000000000000, 4.330127018922196314 ) ) ;
#109472=CARTESIAN_POINT ( 'NONE',  ( 10.64999999999990976, 2.500000000000000000, -6.248780366869526759 ) ) ;
#109473=ORIENTED_EDGE ( 'NONE', *, *, #110819, .T. ) ;
#109475=FACE_OUTER_BOUND ( 'NONE', #7691, .T. ) ;
#109476=CONICAL_SURFACE ( 'NONE', #82298, 0.1000000000000002554, 0.003490658503988666988 ) ;
#109477=DIRECTION ( 'NONE',  ( 0.000000000000000000, 0.000000000000000000, 1.000000000000000000 ) ) ;
#109478=AXIS2_PLACEMENT_3D ( 'NONE', #71558, #1524, #51303 ) ;
#109479=VECTOR ( 'NONE', #75072, 1000.000000000000000 ) ;
#109480=DIRECTION ( 'NONE',  ( -0.000000000000000000, -1.000000000000000000, -0.000000000000000000 ) ) ;
#109481=CARTESIAN_POINT ( 'NONE',  ( 13.34999999999990017, 12.50000000000000000, 1.537336459617582918 ) ) ;
#109482=CARTESIAN_POINT ( 'NONE',  ( 9.399999999999915090, 2.500000000000000000, 4.676537180435972552 ) ) ;
#109483=CIRCLE ( 'NONE', #126207, 0.06509327318403745899 ) ;
#109484=CARTESIAN_POINT ( 'NONE',  ( 5.199999999999931788, 2.500000000000000000, 4.576537180435972019 ) ) ;
#109485=AXIS2_PLACEMENT_3D ( 'NONE', #44761, #74860, #13343 ) ;
#109486=VERTEX_POINT ( 'NONE', #9465 ) ;
#109487=ORIENTED_EDGE ( 'NONE', *, *, #104925, .F. ) ;
#109488=VERTEX_POINT ( 'NONE', #12030 ) ;
#109489=ORIENTED_EDGE ( 'NONE', *, *, #61233, .F. ) ;
#109490=DIRECTION ( 'NONE',  ( 0.000000000000000000, 1.000000000000000000, 0.000000000000000000 ) ) ;
#109491=DIRECTION ( 'NONE',  ( 0.000000000000000000, 1.000000000000000000, 0.000000000000000000 ) ) ;
#109492=DIRECTION ( 'NONE',  ( 0.000000000000000000, 0.000000000000000000, -1.000000000000000000 ) ) ;
#109493=ORIENTED_EDGE ( 'NONE', *, *, #97697, .T. ) ;
#109494=FACE_BOUND ( 'NONE', #94852, .T. ) ;
#109495=VERTEX_POINT ( 'NONE', #266 ) ;
#109496=DIRECTION ( 'NONE',  ( -0.000000000000000000, -1.000000000000000000, -0.000000000000000000 ) ) ;
#109497=DIRECTION ( 'NONE',  ( 0.000000000000000000, 0.000000000000000000, -1.000000000000000000 ) ) ;
#109499=FACE_OUTER_BOUND ( 'NONE', #88807, .T. ) ;
#109500=DIRECTION ( 'NONE',  ( 0.000000000000000000, 0.000000000000000000, 1.000000000000000000 ) ) ;
#109501=CARTESIAN_POINT ( 'NONE',  ( -9.600000000000008527, 2.500000000000000000, -3.537306695894645969 ) ) ;
#109502=VERTEX_POINT ( 'NONE', #80143 ) ;
#109503=DIRECTION ( 'NONE',  ( 0.000000000000000000, -0.9999939076577903929, 0.003490651415223739937 ) ) ;
#109504=AXIS2_PLACEMENT_3D ( 'NONE', #121083, #21596, #92255 ) ;
#109505=DIRECTION ( 'NONE',  ( -0.000000000000000000, 1.000000000000000000, -0.000000000000000000 ) ) ;
#109506=PLANE ( 'NONE',  #91995 ) ;
#109507=EDGE_CURVE ( 'NONE', #26903, #64905, #65728, .T. ) ;
#109508=VECTOR ( 'NONE', #51983, 1000.000000000000000 ) ;
#109509=CONICAL_SURFACE ( 'NONE', #126231, 0.1000000000000002554, 0.003490658503988666988 ) ;
#109510=VERTEX_POINT ( 'NONE', #51979 ) ;
#109511=ORIENTED_EDGE ( 'NONE', *, *, #98125, .F. ) ;
#109512=ORIENTED_EDGE ( 'NONE', *, *, #45289, .T. ) ;
#109513=AXIS2_PLACEMENT_3D ( 'NONE', #51966, #120692, #915 ) ;
#109514=EDGE_LOOP ( 'NONE', ( #64051, #24100, #83390, #102365 ) ) ;
#109515=DIRECTION ( 'NONE',  ( 0.000000000000000000, 1.000000000000000000, 0.000000000000000000 ) ) ;
#109516=AXIS2_PLACEMENT_3D ( 'NONE', #17414, #57361, #97282 ) ;
#109517=CIRCLE ( 'NONE', #52784, 0.1000000000000000472 ) ;
#109518=DIRECTION ( 'NONE',  ( 0.000000000000000000, 0.000000000000000000, -1.000000000000000000 ) ) ;
#109519=VERTEX_POINT ( 'NONE', #91893 ) ;
#109520=ORIENTED_EDGE ( 'NONE', *, *, #49242, .F. ) ;
#109521=ORIENTED_EDGE ( 'NONE', *, *, #22000, .T. ) ;
#109522=CARTESIAN_POINT ( 'NONE',  ( 14.14999999999989733, 2.500000000000000000, 1.572243186433545548 ) ) ;
#109523=EDGE_CURVE ( 'NONE', #72018, #125678, #86660, .T. ) ;
#109524=AXIS2_PLACEMENT_3D ( 'NONE', #101389, #94778, #105240 ) ;
#109525=CIRCLE ( 'NONE', #84479, 0.1000000000000000472 ) ;
#109526=CIRCLE ( 'NONE', #53087, 0.1000000000000002554 ) ;
#109527=CARTESIAN_POINT ( 'NONE',  ( 4.349999999999939249, 12.50000000000000000, 2.511473670974873507 ) ) ;
#109528=FACE_OUTER_BOUND ( 'NONE', #14134, .T. ) ;
#109529=DIRECTION ( 'NONE',  ( 0.000000000000000000, 1.000000000000000000, 0.000000000000000000 ) ) ;
#109530=DIRECTION ( 'NONE',  ( -0.000000000000000000, 1.000000000000000000, -0.000000000000000000 ) ) ;
#109531=PLANE ( 'NONE',  #51885 ) ;
#109532=VECTOR ( 'NONE', #100216, 1000.000000000000000 ) ;
#109533=EDGE_CURVE ( 'NONE', #125468, #70303, #76211, .T. ) ;
#109534=CARTESIAN_POINT ( 'NONE',  ( -4.800000000000024691, 2.500000000000000000, 4.576537180435972019 ) ) ;
#109535=EDGE_CURVE ( 'NONE', #25981, #37478, #5085, .T. ) ;
#109536=ORIENTED_EDGE ( 'NONE', *, *, #107218, .F. ) ;
#109537=CARTESIAN_POINT ( 'NONE',  ( -3.350000000000028511, 2.500000000000000000, 1.572243186433545548 ) ) ;
#109539=ORIENTED_EDGE ( 'NONE', *, *, #54304, .T. ) ;
#109541=CARTESIAN_POINT ( 'NONE',  ( 6.449999999999933564, 12.50000000000000000, -6.841600689897078702 ) ) ;
#109542=ORIENTED_EDGE ( 'NONE', *, *, #99287, .T. ) ;
#109543=EDGE_CURVE ( 'NONE', #83720, #87809, #99196, .T. ) ;
#109545=CIRCLE ( 'NONE', #875, 0.09999999999999982514 ) ;
#109546=FACE_OUTER_BOUND ( 'NONE', #79379, .T. ) ;
#109547=CARTESIAN_POINT ( 'NONE',  ( -8.750000000000012434, 2.500000000000000000, -5.802370205355744659 ) ) ;
#109548=LINE ( 'NONE', #50612, #4016 ) ;
#109549=CARTESIAN_POINT ( 'NONE',  ( 1.649999999999951505, 12.50000000000000000, -1.537336459617587581 ) ) ;
#109550=DIRECTION ( 'NONE',  ( 0.000000000000000000, 1.000000000000000000, 0.000000000000000000 ) ) ;
#109551=VERTEX_POINT ( 'NONE', #123916 ) ;
#109552=CARTESIAN_POINT ( 'NONE',  ( 2.899999999999946620, 2.500000000000000000, -5.122947341949753763 ) ) ;
#109553=AXIS2_PLACEMENT_3D ( 'NONE', #122216, #52817, #12868 ) ;
#109554=AXIS2_PLACEMENT_3D ( 'NONE', #62926, #24939, #43308 ) ;
#109555=ORIENTED_EDGE ( 'NONE', *, *, #58446, .F. ) ;
#109556=DIRECTION ( 'NONE',  ( -0.000000000000000000, 1.000000000000000000, -0.000000000000000000 ) ) ;
#109557=EDGE_LOOP ( 'NONE', ( #73901, #82508, #37933, #91542 ) ) ;
#109558=DIRECTION ( 'NONE',  ( 0.000000000000000000, 0.000000000000000000, -1.000000000000000000 ) ) ;
#109559=FACE_OUTER_BOUND ( 'NONE', #110976, .T. ) ;
#109560=VERTEX_POINT ( 'NONE', #34279 ) ;
#109561=FACE_OUTER_BOUND ( 'NONE', #61845, .T. ) ;
#109562=DIRECTION ( 'NONE',  ( 0.000000000000000000, 1.000000000000000000, 0.000000000000000000 ) ) ;
#109563=ORIENTED_EDGE ( 'NONE', *, *, #97152, .F. ) ;
#109564=VECTOR ( 'NONE', #126593, 1000.000000000000000 ) ;
#109565=AXIS2_PLACEMENT_3D ( 'NONE', #33137, #5571, #33759 ) ;
#109566=EDGE_CURVE ( 'NONE', #100401, #109850, #74050, .T. ) ;
#109567=DIRECTION ( 'NONE',  ( -0.000000000000000000, 1.000000000000000000, -0.000000000000000000 ) ) ;
#109568=ORIENTED_EDGE ( 'NONE', *, *, #79414, .F. ) ;
#109570=DIRECTION ( 'NONE',  ( 0.000000000000000000, -0.000000000000000000, 1.000000000000000000 ) ) ;
#109571=DIRECTION ( 'NONE',  ( -0.000000000000000000, 1.000000000000000000, -0.000000000000000000 ) ) ;
#109572=EDGE_CURVE ( 'NONE', #122791, #91186, #90768, .T. ) ;
#109573=DIRECTION ( 'NONE',  ( 0.000000000000000000, 0.000000000000000000, 1.000000000000000000 ) ) ;
#109574=DIRECTION ( 'NONE',  ( -0.000000000000000000, 1.000000000000000000, -0.000000000000000000 ) ) ;
#109575=EDGE_CURVE ( 'NONE', #80133, #26576, #78278, .T. ) ;
#109576=DIRECTION ( 'NONE',  ( 0.000000000000000000, 1.000000000000000000, 0.000000000000000000 ) ) ;
#109577=EDGE_LOOP ( 'NONE', ( #1911, #120337 ) ) ;
#109578=CIRCLE ( 'NONE', #38585, 0.1000000000000002554 ) ;
#109579=CONICAL_SURFACE ( 'NONE', #92858, 0.1000000000000002554, 0.003490658503988666988 ) ;
#109580=CIRCLE ( 'NONE', #67703, 0.06509327318403745899 ) ;
#109581=DIRECTION ( 'NONE',  ( -0.000000000000000000, 1.000000000000000000, -0.000000000000000000 ) ) ;
#109582=EDGE_CURVE ( 'NONE', #42734, #3753, #25082, .T. ) ;
#109583=ADVANCED_FACE ( 'NONE', ( #64985 ), #109749, .T. ) ;
#109584=EDGE_CURVE ( 'NONE', #46350, #94980, #15235, .T. ) ;
#109585=EDGE_CURVE ( 'NONE', #77027, #102170, #32412, .T. ) ;
#109587=CIRCLE ( 'NONE', #117882, 0.1000000000000002554 ) ;
#109588=CARTESIAN_POINT ( 'NONE',  ( -0.6500000000000398792, 2.500000000000000000, -6.741600689897078169 ) ) ;
#109589=CARTESIAN_POINT ( 'NONE',  ( -4.200000000000029488, 2.500000000000000000, -4.330127018922201643 ) ) ;
#109590=ADVANCED_FACE ( 'NONE', ( #53902 ), #9404, .T. ) ;
#109591=DIRECTION ( 'NONE',  ( 0.000000000000000000, 0.000000000000000000, -1.000000000000000000 ) ) ;
#109592=DIRECTION ( 'NONE',  ( -0.000000000000000000, 1.000000000000000000, -0.000000000000000000 ) ) ;
#109593=DIRECTION ( 'NONE',  ( 0.000000000000000000, 0.000000000000000000, -1.000000000000000000 ) ) ;
#109594=CARTESIAN_POINT ( 'NONE',  ( 14.14999999999989377, 2.500000000000000000, -1.572243186433550211 ) ) ;
#109595=FACE_OUTER_BOUND ( 'NONE', #91110, .T. ) ;
#109596=ORIENTED_EDGE ( 'NONE', *, *, #83554, .F. ) ;
#109597=EDGE_CURVE ( 'NONE', #8654, #43734, #55363, .T. ) ;
#109598=CARTESIAN_POINT ( 'NONE',  ( -14.59999999999998366, 2.500000000000000000, -1.084202172485504434E-16 ) ) ;
#109599=DIRECTION ( 'NONE',  ( 0.000000000000000000, 1.000000000000000000, 0.000000000000000000 ) ) ;
#109600=DIRECTION ( 'NONE',  ( 0.000000000000000000, 0.000000000000000000, -1.000000000000000000 ) ) ;
#109601=CONICAL_SURFACE ( 'NONE', #117987, 0.1000000000000002554, 0.003490658503988666988 ) ;
#109602=AXIS2_PLACEMENT_3D ( 'NONE', #115645, #64621, #126776 ) ;
#109603=AXIS2_PLACEMENT_3D ( 'NONE', #97415, #77763, #58792 ) ;
#109604=ORIENTED_EDGE ( 'NONE', *, *, #56730, .F. ) ;
#109605=DIRECTION ( 'NONE',  ( 0.000000000000000000, 1.000000000000000000, 0.000000000000000000 ) ) ;
#109606=VECTOR ( 'NONE', #107513, 1000.000000000000000 ) ;
#109607=VECTOR ( 'NONE', #101977, 1000.000000000000000 ) ;
#109608=ORIENTED_EDGE ( 'NONE', *, *, #128005, .T. ) ;
#109609=CONICAL_SURFACE ( 'NONE', #51130, 0.09999999999999999167, 0.003490658503988666988 ) ;
#109610=ORIENTED_EDGE ( 'NONE', *, *, #105764, .F. ) ;
#109611=DIRECTION ( 'NONE',  ( -0.000000000000000000, 1.000000000000000000, -0.000000000000000000 ) ) ;
#109612=ORIENTED_EDGE ( 'NONE', *, *, #17046, .F. ) ;
#109613=DIRECTION ( 'NONE',  ( 0.000000000000000000, 1.000000000000000000, 0.000000000000000000 ) ) ;
#109614=CARTESIAN_POINT ( 'NONE',  ( -11.25000000000000000, 2.500000000000000000, 7.188010851410848723 ) ) ;
#109615=AXIS2_PLACEMENT_3D ( 'NONE', #117605, #27971, #58089 ) ;
#109616=VERTEX_POINT ( 'NONE', #34925 ) ;
#109617=AXIS2_PLACEMENT_3D ( 'NONE', #90212, #111138, #43097 ) ;
#109618=CIRCLE ( 'NONE', #46834, 0.1000000000000002554 ) ;
#109619=DIRECTION ( 'NONE',  ( -4.274815082592931898E-19, -0.9999939076577903929, -0.003490651415223739937 ) ) ;
#109620=FACE_OUTER_BOUND ( 'NONE', #2889, .T. ) ;
#109621=AXIS2_PLACEMENT_3D ( 'NONE', #128249, #66079, #86357 ) ;
#109622=FACE_OUTER_BOUND ( 'NONE', #72865, .T. ) ;
#109623=VERTEX_POINT ( 'NONE', #93826 ) ;
#109624=EDGE_CURVE ( 'NONE', #118224, #87786, #11445, .T. ) ;
#109626=ORIENTED_EDGE ( 'NONE', *, *, #37624, .T. ) ;
#109627=DIRECTION ( 'NONE',  ( 0.000000000000000000, -0.000000000000000000, 1.000000000000000000 ) ) ;
#109629=DIRECTION ( 'NONE',  ( -0.000000000000000000, -1.000000000000000000, -0.000000000000000000 ) ) ;
#109630=FACE_BOUND ( 'NONE', #104780, .T. ) ;
#109631=EDGE_LOOP ( 'NONE', ( #107153, #6607 ) ) ;
#109632=DIRECTION ( 'NONE',  ( 0.000000000000000000, 0.000000000000000000, 1.000000000000000000 ) ) ;
#109633=CARTESIAN_POINT ( 'NONE',  ( 12.29999999999990656, 2.500000000000000000, -4.776537180435977525 ) ) ;
#109634=VECTOR ( 'NONE', #44044, 1000.000000000000000 ) ;
#109635=ORIENTED_EDGE ( 'NONE', *, *, #48656, .F. ) ;
#109636=EDGE_CURVE ( 'NONE', #94218, #59296, #30349, .T. ) ;
#109637=CARTESIAN_POINT ( 'NONE',  ( -8.750000000000008882, 2.500000000000000000, -2.757883832488654097 ) ) ;
#109638=DIRECTION ( 'NONE',  ( 0.000000000000000000, 0.000000000000000000, 1.000000000000000000 ) ) ;
#109639=DIRECTION ( 'NONE',  ( -4.274815082592931898E-19, -0.9999939076577903929, -0.003490651415223739937 ) ) ;
#109640=DIRECTION ( 'NONE',  ( -0.000000000000000000, 1.000000000000000000, -0.000000000000000000 ) ) ;
#109641=DIRECTION ( 'NONE',  ( 0.000000000000000000, 0.000000000000000000, 1.000000000000000000 ) ) ;
#109642=CARTESIAN_POINT ( 'NONE',  ( 8.749999999999957367, 12.50000000000000000, -6.495190528383302464 ) ) ;
#109643=DIRECTION ( 'NONE',  ( -4.274815082592931898E-19, -0.9999939076577903929, -0.003490651415223739937 ) ) ;
#109644=AXIS2_PLACEMENT_3D ( 'NONE', #98521, #78281, #67790 ) ;
#109645=CONICAL_SURFACE ( 'NONE', #69935, 0.09999999999999982514, 0.003490658503988666988 ) ;
#109646=VERTEX_POINT ( 'NONE', #44077 ) ;
#109647=VERTEX_POINT ( 'NONE', #13313 ) ;
#109648=ORIENTED_EDGE ( 'NONE', *, *, #90938, .F. ) ;
#109649=ORIENTED_EDGE ( 'NONE', *, *, #115871, .F. ) ;
#109650=ORIENTED_EDGE ( 'NONE', *, *, #84854, .T. ) ;
#109651=DIRECTION ( 'NONE',  ( 0.000000000000000000, 1.000000000000000000, 0.000000000000000000 ) ) ;
#109652=DIRECTION ( 'NONE',  ( -0.000000000000000000, -1.000000000000000000, -0.000000000000000000 ) ) ;
#109653=ORIENTED_EDGE ( 'NONE', *, *, #39200, .T. ) ;
#109654=FACE_BOUND ( 'NONE', #93684, .T. ) ;
#109655=DIRECTION ( 'NONE',  ( 0.000000000000000000, -0.9999939076577903929, 0.003490651415223739937 ) ) ;
#109656=CIRCLE ( 'NONE', #103307, 0.1000000000000002554 ) ;
#109657=FACE_OUTER_BOUND ( 'NONE', #37725, .T. ) ;
#109658=CONICAL_SURFACE ( 'NONE', #28181, 0.1000000000000002554, 0.003490658503988666988 ) ;
#109659=CARTESIAN_POINT ( 'NONE',  ( -2.900000000000029221, 2.500000000000000000, -0.6928203230275541413 ) ) ;
#109661=DIRECTION ( 'NONE',  ( 0.000000000000000000, 0.000000000000000000, -1.000000000000000000 ) ) ;
#109662=DIRECTION ( 'NONE',  ( -0.000000000000000000, -1.000000000000000000, -0.000000000000000000 ) ) ;
#109663=ORIENTED_EDGE ( 'NONE', *, *, #89463, .T. ) ;
#109664=ORIENTED_EDGE ( 'NONE', *, *, #20445, .T. ) ;
#109665=ADVANCED_FACE ( 'NONE', ( #123285 ), #30255, .T. ) ;
#109666=CONICAL_SURFACE ( 'NONE', #55378, 0.09999999999999982514, 0.003490658503988666988 ) ;
#109667=VERTEX_POINT ( 'NONE', #24441 ) ;
#109668=EDGE_LOOP ( 'NONE', ( #89607, #85863, #3799, #115478 ) ) ;
#109669=CIRCLE ( 'NONE', #13500, 0.1000000000000002554 ) ;
#109670=ORIENTED_EDGE ( 'NONE', *, *, #39439, .F. ) ;
#109671=ORIENTED_EDGE ( 'NONE', *, *, #99074, .T. ) ;
#109672=CARTESIAN_POINT ( 'NONE',  ( 15.40585131959762499, 2.499999999999999112, 5.817868759122426958 ) ) ;
#109673=LINE ( 'NONE', #119471, #80236 ) ;
#109674=AXIS2_PLACEMENT_3D ( 'NONE', #83882, #16408, #76000 ) ;
#109675=EDGE_LOOP ( 'NONE', ( #95184, #87236, #102717, #112940 ) ) ;
#109676=DIRECTION ( 'NONE',  ( 0.000000000000000000, -0.9999939076577903929, 0.003490651415223739937 ) ) ;
#109677=CIRCLE ( 'NONE', #78296, 0.06509327318403745899 ) ;
#109678=EDGE_CURVE ( 'NONE', #99929, #24133, #21929, .T. ) ;
#109679=FACE_OUTER_BOUND ( 'NONE', #34475, .T. ) ;
#109680=CARTESIAN_POINT ( 'NONE',  ( 3.549999999999943867, 12.50000000000000000, -6.148780366869526226 ) ) ;
#109683=CARTESIAN_POINT ( 'NONE',  ( 2.949999999999946887, 12.50000000000000000, -2.230156782645139391 ) ) ;
#109684=EDGE_CURVE ( 'NONE', #95907, #6696, #90868, .T. ) ;
#109685=DIRECTION ( 'NONE',  ( 0.000000000000000000, 0.000000000000000000, -1.000000000000000000 ) ) ;
#109686=EDGE_CURVE ( 'NONE', #36888, #117215, #15632, .T. ) ;
#109688=LINE ( 'NONE', #27241, #27464 ) ;
#109690=VERTEX_POINT ( 'NONE', #83369 ) ;
#109691=CARTESIAN_POINT ( 'NONE',  ( 14.34999999999989306, 2.500000000000000000, -1.918653347947326004 ) ) ;
#109692=ADVANCED_FACE ( 'NONE', ( #73523 ), #72099, .T. ) ;
#109693=CIRCLE ( 'NONE', #28211, 0.06509327318403741736 ) ;
#109694=CIRCLE ( 'NONE', #62900, 0.06509327318403745899 ) ;
#109695=CARTESIAN_POINT ( 'NONE',  ( 2.049999999999950084, 12.50000000000000000, -2.230156782645139391 ) ) ;
#109696=AXIS2_PLACEMENT_3D ( 'NONE', #51893, #33546, #62985 ) ;
#109697=DIRECTION ( 'NONE',  ( 0.000000000000000000, 0.000000000000000000, 1.000000000000000000 ) ) ;
#109698=EDGE_CURVE ( 'NONE', #15257, #9179, #74150, .T. ) ;
#109699=ORIENTED_EDGE ( 'NONE', *, *, #107527, .F. ) ;
#109700=VERTEX_POINT ( 'NONE', #56462 ) ;
#109701=DIRECTION ( 'NONE',  ( -4.274815082592931898E-19, -0.9999939076577903929, -0.003490651415223739937 ) ) ;
#109702=CIRCLE ( 'NONE', #126423, 0.06509327318403741736 ) ;
#109703=CIRCLE ( 'NONE', #26078, 0.06509327318403743123 ) ;
#109704=CARTESIAN_POINT ( 'NONE',  ( -12.29999999999999538, 12.50000000000000000, 4.741630453620009789 ) ) ;
#109705=CARTESIAN_POINT ( 'NONE',  ( -7.500000000000016875, 12.50000000000000000, 0.6928203230275494784 ) ) ;
#109706=DIRECTION ( 'NONE',  ( 0.000000000000000000, -0.000000000000000000, 1.000000000000000000 ) ) ;
#109707=ORIENTED_EDGE ( 'NONE', *, *, #50320, .F. ) ;
#109708=AXIS2_PLACEMENT_3D ( 'NONE', #94123, #82390, #35224 ) ;
#109709=DIRECTION ( 'NONE',  ( 0.000000000000000000, -0.000000000000000000, 1.000000000000000000 ) ) ;
#109710=ORIENTED_EDGE ( 'NONE', *, *, #9967, .T. ) ;
#109711=CARTESIAN_POINT ( 'NONE',  ( -5.450000000000019718, 12.50000000000000000, 2.099970236277060032 ) ) ;
#109712=CIRCLE ( 'NONE', #97178, 0.1000000000000000472 ) ;
#109713=AXIS2_PLACEMENT_3D ( 'NONE', #1931, #72627, #101437 ) ;
#109714=VERTEX_POINT ( 'NONE', #96382 ) ;
#109715=CARTESIAN_POINT ( 'NONE',  ( -13.74999999999998934, 2.500000000000000000, -1.572243186433547990 ) ) ;
#109716=DIRECTION ( 'NONE',  ( 0.000000000000000000, 0.000000000000000000, 1.000000000000000000 ) ) ;
#109717=DIRECTION ( 'NONE',  ( -0.000000000000000000, -1.000000000000000000, -0.000000000000000000 ) ) ;
#109718=AXIS2_PLACEMENT_3D ( 'NONE', #122933, #73812, #54191 ) ;
#109719=CARTESIAN_POINT ( 'NONE',  ( -10.20000000000000284, 2.500000000000000000, -0.3464101615137782364 ) ) ;
#109720=VERTEX_POINT ( 'NONE', #106226 ) ;
#109721=CARTESIAN_POINT ( 'NONE',  ( -13.34999999999999076, 2.500000000000000000, -2.165063509461099489 ) ) ;
#109722=VERTEX_POINT ( 'NONE', #126510 ) ;
#109723=EDGE_LOOP ( 'NONE', ( #83859, #84628 ) ) ;
#109724=DIRECTION ( 'NONE',  ( -4.274815082592931898E-19, -0.9999939076577903929, -0.003490651415223739937 ) ) ;
#109725=CARTESIAN_POINT ( 'NONE',  ( 97.50000000000000000, -1.500000000000000222, -1.322875655532295136 ) ) ;
#109726=DIRECTION ( 'NONE',  ( 0.000000000000000000, -0.000000000000000000, 1.000000000000000000 ) ) ;
#109728=DIRECTION ( 'NONE',  ( -0.000000000000000000, -1.000000000000000000, -0.000000000000000000 ) ) ;
#109729=FACE_OUTER_BOUND ( 'NONE', #12339, .T. ) ;
#109730=CARTESIAN_POINT ( 'NONE',  ( 5.849999999999935696, 2.500000000000000000, -6.395190528383301931 ) ) ;
#109731=DIRECTION ( 'NONE',  ( -0.000000000000000000, -1.000000000000000000, -0.000000000000000000 ) ) ;
#109732=DIRECTION ( 'NONE',  ( 0.000000000000000000, -0.000000000000000000, 1.000000000000000000 ) ) ;
#109733=EDGE_CURVE ( 'NONE', #46924, #129420, #107509, .T. ) ;
#109734=EDGE_CURVE ( 'NONE', #70361, #94856, #42876, .T. ) ;
#109735=EDGE_CURVE ( 'NONE', #19417, #52442, #13582, .T. ) ;
#109736=CONICAL_SURFACE ( 'NONE', #70028, 0.09999999999999982514, 0.003490658503988666988 ) ;
#109737=EDGE_CURVE ( 'NONE', #63445, #22700, #76117, .T. ) ;
#109738=CONICAL_SURFACE ( 'NONE', #40805, 0.1000000000000000472, 0.003490658503988666988 ) ;
#109739=EDGE_LOOP ( 'NONE', ( #111345, #88578 ) ) ;
#109740=EDGE_CURVE ( 'NONE', #65438, #82940, #120120, .T. ) ;
#109741=LINE ( 'NONE', #10856, #57045 ) ;
#109742=CARTESIAN_POINT ( 'NONE',  ( -1.700000000000034817, 2.500000000000000000, -4.330127018922201643 ) ) ;
#109743=FACE_OUTER_BOUND ( 'NONE', #126045, .T. ) ;
#109744=CARTESIAN_POINT ( 'NONE',  ( -12.69999999999999218, 2.500000000000000000, -4.676537180435975216 ) ) ;
#109745=DIRECTION ( 'NONE',  ( -0.000000000000000000, 1.000000000000000000, -0.000000000000000000 ) ) ;
#109746=ORIENTED_EDGE ( 'NONE', *, *, #118116, .T. ) ;
#109747=ADVANCED_FACE ( 'NONE', ( #117289 ), #34448, .T. ) ;
#109748=FACE_OUTER_BOUND ( 'NONE', #72334, .T. ) ;
#109749=CONICAL_SURFACE ( 'NONE', #46968, 0.1000000000000002554, 0.003490658503988666988 ) ;
#109750=ADVANCED_FACE ( 'NONE', ( #57774 ), #63692, .T. ) ;
#109751=AXIS2_PLACEMENT_3D ( 'NONE', #75196, #73903, #105302 ) ;
#109752=DIRECTION ( 'NONE',  ( 0.000000000000000000, -0.000000000000000000, 1.000000000000000000 ) ) ;
#109753=LINE ( 'NONE', #20084, #98529 ) ;
#109754=ORIENTED_EDGE ( 'NONE', *, *, #87969, .T. ) ;
#109755=ORIENTED_EDGE ( 'NONE', *, *, #43878, .T. ) ;
#109756=CARTESIAN_POINT ( 'NONE',  ( 3.299999999999944755, 2.500000000000000000, -4.430127018922202176 ) ) ;
#109757=AXIS2_PLACEMENT_3D ( 'NONE', #296, #120103, #114141 ) ;
#109758=CONICAL_SURFACE ( 'NONE', #38675, 0.1000000000000002554, 0.003490658503988666988 ) ;
#109759=ORIENTED_EDGE ( 'NONE', *, *, #118271, .T. ) ;
#109760=ORIENTED_EDGE ( 'NONE', *, *, #88062, .T. ) ;
#109761=VERTEX_POINT ( 'NONE', #47955 ) ;
#109762=CARTESIAN_POINT ( 'NONE',  ( -6.650000000000015454, 2.500000000000000000, 2.857883832488649301 ) ) ;
#109763=CARTESIAN_POINT ( 'NONE',  ( -0.6500000000000403233, 12.50000000000000000, 6.083687093685482772 ) ) ;
#109764=FACE_OUTER_BOUND ( 'NONE', #39264, .T. ) ;
#109765=CARTESIAN_POINT ( 'NONE',  ( 2.949999999999946887, 12.50000000000000000, -2.165063509461101710 ) ) ;
#109766=EDGE_LOOP ( 'NONE', ( #96506, #15441, #58131, #31276 ) ) ;
#109767=CARTESIAN_POINT ( 'NONE',  ( -3.550000000000030909, 12.50000000000000000, -6.841600689897078702 ) ) ;
#109768=ORIENTED_EDGE ( 'NONE', *, *, #26978, .T. ) ;
#109769=DIRECTION ( 'NONE',  ( 0.000000000000000000, 0.000000000000000000, 1.000000000000000000 ) ) ;
#109770=CARTESIAN_POINT ( 'NONE',  ( 2.899999999999946620, 2.500000000000000000, -5.022947341949754119 ) ) ;
#109771=CARTESIAN_POINT ( 'NONE',  ( 9.399999999999918643, 2.500000000000000000, -0.3464101615137782364 ) ) ;
#109772=CIRCLE ( 'NONE', #126499, 0.06509327318403745899 ) ;
#109773=ORIENTED_EDGE ( 'NONE', *, *, #116802, .F. ) ;
#109774=ORIENTED_EDGE ( 'NONE', *, *, #20431, .F. ) ;
#109775=ORIENTED_EDGE ( 'NONE', *, *, #87826, .F. ) ;
#109776=AXIS2_PLACEMENT_3D ( 'NONE', #97808, #8133, #29095 ) ;
#109777=VERTEX_POINT ( 'NONE', #75462 ) ;
#109778=ORIENTED_EDGE ( 'NONE', *, *, #53050, .F. ) ;
#109779=DIRECTION ( 'NONE',  ( 0.000000000000000000, 0.000000000000000000, 1.000000000000000000 ) ) ;
#109780=DIRECTION ( 'NONE',  ( 0.000000000000000000, 0.000000000000000000, 1.000000000000000000 ) ) ;
#109781=AXIS2_PLACEMENT_3D ( 'NONE', #24994, #16437, #17066 ) ;
#109782=CARTESIAN_POINT ( 'NONE',  ( 11.44999999999990870, 2.500000000000000000, -1.718653347947326049 ) ) ;
#109783=FACE_BOUND ( 'NONE', #7772, .T. ) ;
#109784=DIRECTION ( 'NONE',  ( 0.000000000000000000, 1.000000000000000000, 0.000000000000000000 ) ) ;
#109786=DIRECTION ( 'NONE',  ( 0.000000000000000000, 0.000000000000000000, 1.000000000000000000 ) ) ;
#109787=CARTESIAN_POINT ( 'NONE',  ( 4.599999999999940137, 2.500000000000000000, -5.122947341949753763 ) ) ;
#109788=AXIS2_PLACEMENT_3D ( 'NONE', #87467, #124838, #24703 ) ;
#109789=ADVANCED_FACE ( 'NONE', ( #68219 ), #84614, .T. ) ;
#109790=AXIS2_PLACEMENT_3D ( 'NONE', #2433, #1162, #21445 ) ;
#109791=CIRCLE ( 'NONE', #40862, 0.06509327318403745899 ) ;
#109792=FACE_OUTER_BOUND ( 'NONE', #72508, .T. ) ;
#109793=CIRCLE ( 'NONE', #128602, 0.09999999999999982514 ) ;
#109794=CARTESIAN_POINT ( 'NONE',  ( -9.350000000000008527, 2.500000000000000000, -6.741600689897071952 ) ) ;
#109795=CARTESIAN_POINT ( 'NONE',  ( -1.900000000000034994, 2.500000000000000000, -4.676537180435978769 ) ) ;
#109796=CIRCLE ( 'NONE', #63830, 0.1000000000000002554 ) ;
#109797=AXIS2_PLACEMENT_3D ( 'NONE', #2255, #93881, #103042 ) ;
#109798=DIRECTION ( 'NONE',  ( 0.000000000000000000, -0.9999939076577903929, 0.003490651415223739937 ) ) ;
#109799=ORIENTED_EDGE ( 'NONE', *, *, #74964, .F. ) ;
#109800=ORIENTED_EDGE ( 'NONE', *, *, #127186, .T. ) ;
#109801=ORIENTED_EDGE ( 'NONE', *, *, #64217, .T. ) ;
#109802=EDGE_LOOP ( 'NONE', ( #78957, #109912 ) ) ;
#109803=CIRCLE ( 'NONE', #116052, 0.06509327318403745899 ) ;
#109804=DIRECTION ( 'NONE',  ( -0.000000000000000000, 1.000000000000000000, -0.000000000000000000 ) ) ;
#109805=LINE ( 'NONE', #98042, #31949 ) ;
#109806=FACE_BOUND ( 'NONE', #129406, .T. ) ;
#109807=LINE ( 'NONE', #99992, #112628 ) ;
#109808=ORIENTED_EDGE ( 'NONE', *, *, #103812, .T. ) ;
#109809=LINE ( 'NONE', #20143, #122037 ) ;
#109810=DIRECTION ( 'NONE',  ( -0.000000000000000000, 1.000000000000000000, -0.000000000000000000 ) ) ;
#109811=CARTESIAN_POINT ( 'NONE',  ( 7.299999999999927880, 2.500000000000000000, -4.676537180435977881 ) ) ;
#109812=CARTESIAN_POINT ( 'NONE',  ( -5.000000000000024869, 2.500000000000000000, -5.022947341949754119 ) ) ;
#109813=VECTOR ( 'NONE', #56354, 1000.000000000000000 ) ;
#109814=EDGE_LOOP ( 'NONE', ( #114026, #41549 ) ) ;
#109815=DIRECTION ( 'NONE',  ( -0.000000000000000000, 1.000000000000000000, -0.000000000000000000 ) ) ;
#109816=VERTEX_POINT ( 'NONE', #35560 ) ;
#109817=ORIENTED_EDGE ( 'NONE', *, *, #11414, .F. ) ;
#109818=CARTESIAN_POINT ( 'NONE',  ( 6.249999999999930722, 2.500000000000000000, 7.188010851410848723 ) ) ;
#109819=DIRECTION ( 'NONE',  ( 0.000000000000000000, 1.000000000000000000, 0.000000000000000000 ) ) ;
#109820=CIRCLE ( 'NONE', #51351, 0.09999999999999982514 ) ;
#109821=ORIENTED_EDGE ( 'NONE', *, *, #2888, .F. ) ;
#109822=AXIS2_PLACEMENT_3D ( 'NONE', #74221, #21912, #23840 ) ;
#109823=VECTOR ( 'NONE', #115564, 1000.000000000000000 ) ;
#109824=ADVANCED_FACE ( 'NONE', ( #127789 ), #113859, .T. ) ;
#109825=CARTESIAN_POINT ( 'NONE',  ( -8.950000000000009948, 2.500000000000000000, 2.511473670974873507 ) ) ;
#109826=DIRECTION ( 'NONE',  ( 0.000000000000000000, 0.000000000000000000, 1.000000000000000000 ) ) ;
#109827=VERTEX_POINT ( 'NONE', #6690 ) ;
#109828=FACE_OUTER_BOUND ( 'NONE', #116721, .T. ) ;
#109829=VERTEX_POINT ( 'NONE', #46660 ) ;
#109830=EDGE_CURVE ( 'NONE', #112785, #41715, #128556, .T. ) ;
#109831=DIRECTION ( 'NONE',  ( 0.000000000000000000, 0.000000000000000000, 1.000000000000000000 ) ) ;
#109832=EDGE_CURVE ( 'NONE', #60441, #10391, #49121, .T. ) ;
#109833=EDGE_LOOP ( 'NONE', ( #16870, #6602 ) ) ;
#109834=CARTESIAN_POINT ( 'NONE',  ( 1.449999999999949551, 2.500000000000000000, 6.741600689897071952 ) ) ;
#109835=CIRCLE ( 'NONE', #122367, 0.06509327318403745899 ) ;
#109836=ORIENTED_EDGE ( 'NONE', *, *, #19615, .F. ) ;
#109838=CARTESIAN_POINT ( 'NONE',  ( 12.89999999999990266, 12.50000000000000000, 5.088040615133786027 ) ) ;
#109839=EDGE_LOOP ( 'NONE', ( #51025, #13879, #102901, #24823 ) ) ;
#109840=CARTESIAN_POINT ( 'NONE',  ( 1.249999999999988898, 2.500000000000000000, -6.495190528383302464 ) ) ;
#109841=CARTESIAN_POINT ( 'NONE',  ( 1.899999999999949507, 12.50000000000000000, 3.983716857408420964 ) ) ;
#109842=EDGE_CURVE ( 'NONE', #12245, #18723, #116677, .T. ) ;
#109843=EDGE_CURVE ( 'NONE', #119953, #62336, #99286, .T. ) ;
#109844=DIRECTION ( 'NONE',  ( -0.000000000000000000, -1.000000000000000000, -0.000000000000000000 ) ) ;
#109845=ADVANCED_FACE ( 'NONE', ( #76766 ), #57113, .T. ) ;
#109846=LINE ( 'NONE', #117699, #88381 ) ;
#109847=ADVANCED_FACE ( 'NONE', ( #87213 ), #28177, .T. ) ;
#109848=ADVANCED_FACE ( 'NONE', ( #79977 ), #20421, .T. ) ;
#109849=FACE_OUTER_BOUND ( 'NONE', #5577, .T. ) ;
#109850=VERTEX_POINT ( 'NONE', #40061 ) ;
#109851=ORIENTED_EDGE ( 'NONE', *, *, #63489, .T. ) ;
#109852=EDGE_LOOP ( 'NONE', ( #86691, #10411, #65967, #68336 ) ) ;
#109853=DIRECTION ( 'NONE',  ( -0.000000000000000000, -1.000000000000000000, -0.000000000000000000 ) ) ;
#109854=AXIS2_PLACEMENT_3D ( 'NONE', #127198, #37527, #105617 ) ;
#109855=CONICAL_SURFACE ( 'NONE', #40921, 0.09999999999999982514, 0.003490658503988666988 ) ;
#109856=DIRECTION ( 'NONE',  ( -0.000000000000000000, 1.000000000000000000, -0.000000000000000000 ) ) ;
#109857=DIRECTION ( 'NONE',  ( 0.000000000000000000, 1.000000000000000000, 0.000000000000000000 ) ) ;
#109858=ORIENTED_EDGE ( 'NONE', *, *, #72783, .T. ) ;
#109859=VERTEX_POINT ( 'NONE', #29588 ) ;
#109861=EDGE_CURVE ( 'NONE', #87809, #44827, #90421, .T. ) ;
#109862=CARTESIAN_POINT ( 'NONE',  ( -0.6500000000000398792, 12.50000000000000000, -2.511473670974877948 ) ) ;
#109863=ORIENTED_EDGE ( 'NONE', *, *, #83385, .T. ) ;
#109864=FACE_OUTER_BOUND ( 'NONE', #79600, .T. ) ;
#109865=DIRECTION ( 'NONE',  ( 0.000000000000000000, -0.000000000000000000, 1.000000000000000000 ) ) ;
#109867=CIRCLE ( 'NONE', #19978, 0.1000000000000000472 ) ;
#109868=FACE_OUTER_BOUND ( 'NONE', #50624, .T. ) ;
#109869=DIRECTION ( 'NONE',  ( 0.000000000000000000, 0.000000000000000000, -1.000000000000000000 ) ) ;
#109870=FACE_OUTER_BOUND ( 'NONE', #60169, .T. ) ;
#109871=AXIS2_PLACEMENT_3D ( 'NONE', #67991, #118384, #37268 ) ;
#109872=CARTESIAN_POINT ( 'NONE',  ( 3.749999999999942268, 2.500000000000000000, -5.802370205355749988 ) ) ;
#109873=ORIENTED_EDGE ( 'NONE', *, *, #18703, .F. ) ;
#109874=VERTEX_POINT ( 'NONE', #119906 ) ;
#109875=DIRECTION ( 'NONE',  ( -0.000000000000000000, 1.000000000000000000, -0.000000000000000000 ) ) ;
#109876=VECTOR ( 'NONE', #63127, 1000.000000000000000 ) ;
#109877=AXIS2_PLACEMENT_3D ( 'NONE', #23118, #63047, #13283 ) ;
#109879=VERTEX_POINT ( 'NONE', #120551 ) ;
#109881=CARTESIAN_POINT ( 'NONE',  ( -3.100000000000028511, 2.500000000000000000, -3.983716857408426293 ) ) ;
#109882=CARTESIAN_POINT ( 'NONE',  ( -15.19999999999998153, 12.50000000000000000, -0.3464101615137759604 ) ) ;
#109883=CONICAL_SURFACE ( 'NONE', #103526, 0.1000000000000002554, 0.003490658503988666988 ) ;
#109885=DIRECTION ( 'NONE',  ( 0.000000000000000000, 1.000000000000000000, 0.000000000000000000 ) ) ;
#109886=FACE_OUTER_BOUND ( 'NONE', #33057, .T. ) ;
#109887=FACE_OUTER_BOUND ( 'NONE', #26595, .T. ) ;
#109888=EDGE_CURVE ( 'NONE', #20699, #29164, #118053, .T. ) ;
#109889=CONICAL_SURFACE ( 'NONE', #80554, 0.1000000000000002554, 0.003490658503988666988 ) ;
#109890=EDGE_CURVE ( 'NONE', #80232, #15598, #5171, .T. ) ;
#109891=EDGE_CURVE ( 'NONE', #27804, #104330, #88907, .T. ) ;
#109892=DIRECTION ( 'NONE',  ( 0.000000000000000000, 0.000000000000000000, 1.000000000000000000 ) ) ;
#109893=AXIS2_PLACEMENT_3D ( 'NONE', #106343, #16652, #96499 ) ;
#109894=VECTOR ( 'NONE', #23053, 1000.000000000000000 ) ;
#109895=EDGE_LOOP ( 'NONE', ( #95124, #118730, #24604, #36825 ) ) ;
#109896=EDGE_CURVE ( 'NONE', #2388, #60152, #107685, .T. ) ;
#109897=AXIS2_PLACEMENT_3D ( 'NONE', #36294, #128550, #116752 ) ;
#109899=ORIENTED_EDGE ( 'NONE', *, *, #54537, .T. ) ;
#109900=EDGE_CURVE ( 'NONE', #115572, #74354, #103588, .T. ) ;
#109901=ORIENTED_EDGE ( 'NONE', *, *, #15334, .T. ) ;
#109902=DIRECTION ( 'NONE',  ( 0.000000000000000000, 0.000000000000000000, 1.000000000000000000 ) ) ;
#109903=DIRECTION ( 'NONE',  ( 0.000000000000000000, 1.000000000000000000, 0.000000000000000000 ) ) ;
#109904=EDGE_CURVE ( 'NONE', #115877, #29350, #71430, .T. ) ;
#109905=ORIENTED_EDGE ( 'NONE', *, *, #66068, .F. ) ;
#109906=EDGE_CURVE ( 'NONE', #123035, #17965, #110086, .T. ) ;
#109908=CARTESIAN_POINT ( 'NONE',  ( -5.850000000000018296, 12.50000000000000000, 1.407149913249508000 ) ) ;
#109909=ADVANCED_FACE ( 'NONE', ( #60979 ), #100892, .T. ) ;
#109910=PLANE ( 'NONE',  #9345 ) ;
#109911=CARTESIAN_POINT ( 'NONE',  ( -11.24999999999996270, 2.500000000000000000, 6.395190528383296602 ) ) ;
#109912=ORIENTED_EDGE ( 'NONE', *, *, #92723, .F. ) ;
#109913=LINE ( 'NONE', #91553, #13976 ) ;
#109914=VECTOR ( 'NONE', #8529, 1000.000000000000000 ) ;
#109915=EDGE_CURVE ( 'NONE', #12077, #1020, #128641, .T. ) ;
#109916=DIRECTION ( 'NONE',  ( -0.000000000000000000, -1.000000000000000000, -0.000000000000000000 ) ) ;
#109917=ORIENTED_EDGE ( 'NONE', *, *, #128230, .T. ) ;
#109918=ORIENTED_EDGE ( 'NONE', *, *, #115388, .F. ) ;
#109919=VERTEX_POINT ( 'NONE', #50510 ) ;
#109920=VERTEX_POINT ( 'NONE', #9305 ) ;
#109921=CARTESIAN_POINT ( 'NONE',  ( -3.750000000000029310, 12.50000000000000000, -7.188010851410854052 ) ) ;
#109922=AXIS2_PLACEMENT_3D ( 'NONE', #77297, #117187, #27534 ) ;
#109923=AXIS2_PLACEMENT_3D ( 'NONE', #10605, #17864, #39478 ) ;
#109924=DIRECTION ( 'NONE',  ( -0.000000000000000000, -1.000000000000000000, -0.000000000000000000 ) ) ;
#109925=CARTESIAN_POINT ( 'NONE',  ( 3.749999999999944045, 12.50000000000000000, -2.922977105672691422 ) ) ;
#109926=CIRCLE ( 'NONE', #61907, 0.1000000000000002554 ) ;
#109927=AXIS2_PLACEMENT_3D ( 'NONE', #90291, #20286, #121061 ) ;
#109928=DIRECTION ( 'NONE',  ( 0.000000000000000000, 0.000000000000000000, 1.000000000000000000 ) ) ;
#109929=ORIENTED_EDGE ( 'NONE', *, *, #57575, .F. ) ;
#109930=CARTESIAN_POINT ( 'NONE',  ( 0.6499999999999543920, 12.50000000000000000, 6.841600689897072485 ) ) ;
#109931=PLANE ( 'NONE',  #41352 ) ;
#109933=DIRECTION ( 'NONE',  ( 0.000000000000000000, 0.000000000000000000, 1.000000000000000000 ) ) ;
#109934=ADVANCED_FACE ( 'NONE', ( #31530 ), #124413, .T. ) ;
#109935=AXIS2_PLACEMENT_3D ( 'NONE', #87058, #115881, #66132 ) ;
#109936=VERTEX_POINT ( 'NONE', #109442 ) ;
#109937=CARTESIAN_POINT ( 'NONE',  ( 9.599999999999914380, 12.50000000000000000, 4.395220292106234439 ) ) ;
#109938=CIRCLE ( 'NONE', #86932, 0.1000000000000000056 ) ;
#109939=CONICAL_SURFACE ( 'NONE', #40999, 0.09999999999999999167, 0.003490658503988666988 ) ;
#109940=VERTEX_POINT ( 'NONE', #767 ) ;
#109941=VERTEX_POINT ( 'NONE', #41368 ) ;
#109942=DIRECTION ( 'NONE',  ( 0.000000000000000000, -0.9999939076577903929, 0.003490651415223739937 ) ) ;
#109943=DIRECTION ( 'NONE',  ( 0.000000000000000000, 1.000000000000000000, 0.000000000000000000 ) ) ;
#109944=FACE_BOUND ( 'NONE', #107050, .T. ) ;
#109945=CARTESIAN_POINT ( 'NONE',  ( 9.349999999999919709, 2.500000000000000000, 2.611473670974873151 ) ) ;
#109946=CARTESIAN_POINT ( 'NONE',  ( -10.65000000000000213, 12.50000000000000000, 6.148780366869520009 ) ) ;
#109947=DIRECTION ( 'NONE',  ( 0.000000000000000000, 1.000000000000000000, 0.000000000000000000 ) ) ;
#109948=AXIS2_PLACEMENT_3D ( 'NONE', #58938, #128341, #20301 ) ;
#109949=AXIS2_PLACEMENT_3D ( 'NONE', #34830, #74732, #24984 ) ;
#109950=EDGE_CURVE ( 'NONE', #4680, #1374, #11535, .T. ) ;
#109951=DIRECTION ( 'NONE',  ( 0.000000000000000000, 0.000000000000000000, -1.000000000000000000 ) ) ;
#109952=CARTESIAN_POINT ( 'NONE',  ( -9.150000000000009237, 2.500000000000000000, -1.472243186433550122 ) ) ;
#109953=DIRECTION ( 'NONE',  ( 0.000000000000000000, 0.000000000000000000, 1.000000000000000000 ) ) ;
#109954=DIRECTION ( 'NONE',  ( 0.000000000000000000, 0.000000000000000000, -1.000000000000000000 ) ) ;
#109955=ORIENTED_EDGE ( 'NONE', *, *, #81856, .T. ) ;
#109956=CARTESIAN_POINT ( 'NONE',  ( -13.74999999999995381, 2.500000000000000000, -2.165063509461099489 ) ) ;
#109957=LINE ( 'NONE', #80505, #72520 ) ;
#109958=ORIENTED_EDGE ( 'NONE', *, *, #65950, .T. ) ;
#109959=ORIENTED_EDGE ( 'NONE', *, *, #29162, .T. ) ;
#109960=DIRECTION ( 'NONE',  ( 0.000000000000000000, 0.000000000000000000, -1.000000000000000000 ) ) ;
#109961=EDGE_CURVE ( 'NONE', #111598, #25747, #81277, .T. ) ;
#109962=CARTESIAN_POINT ( 'NONE',  ( 9.999999999999911182, 2.500000000000000000, 5.022947341949748790 ) ) ;
#109963=FACE_BOUND ( 'NONE', #128543, .T. ) ;
#109964=DIRECTION ( 'NONE',  ( 0.000000000000000000, -0.9999939076577903929, 0.003490651415223739937 ) ) ;
#109965=AXIS2_PLACEMENT_3D ( 'NONE', #5341, #55737, #35468 ) ;
#109966=CARTESIAN_POINT ( 'NONE',  ( 2.899999999999944844, 12.50000000000000000, 5.022947341949748790 ) ) ;
#109967=VECTOR ( 'NONE', #5877, 1000.000000000000000 ) ;
#109968=VERTEX_POINT ( 'NONE', #111350 ) ;
#109969=CARTESIAN_POINT ( 'NONE',  ( -3.550000000000027800, 2.500000000000000000, 6.148780366869520009 ) ) ;
#109971=ORIENTED_EDGE ( 'NONE', *, *, #107143, .F. ) ;
#109972=FACE_OUTER_BOUND ( 'NONE', #48840, .T. ) ;
#109974=AXIS2_PLACEMENT_3D ( 'NONE', #68568, #100601, #69873 ) ;
#109975=CARTESIAN_POINT ( 'NONE',  ( 9.799999999999913669, 2.500000000000000000, -4.083716857408426826 ) ) ;
#109976=CARTESIAN_POINT ( 'NONE',  ( 6.049999999999935874, 2.500000000000000000, -6.941600689897077459 ) ) ;
#109977=AXIS2_PLACEMENT_3D ( 'NONE', #63045, #102958, #93161 ) ;
#109978=ORIENTED_EDGE ( 'NONE', *, *, #129344, .F. ) ;
#109979=VECTOR ( 'NONE', #41289, 1000.000000000000000 ) ;
#109980=EDGE_CURVE ( 'NONE', #35273, #25034, #36688, .T. ) ;
#109981=CARTESIAN_POINT ( 'NONE',  ( -12.49999999999995914, 2.500000000000000000, 1.843143693225357538E-15 ) ) ;
#109982=FACE_OUTER_BOUND ( 'NONE', #9851, .T. ) ;
#109983=DIRECTION ( 'NONE',  ( 0.000000000000000000, 1.000000000000000000, 0.000000000000000000 ) ) ;
#109984=LINE ( 'NONE', #103224, #21953 ) ;
#109985=VERTEX_POINT ( 'NONE', #116 ) ;
#109986=ORIENTED_EDGE ( 'NONE', *, *, #91397, .T. ) ;
#109987=DIRECTION ( 'NONE',  ( -0.000000000000000000, 1.000000000000000000, -0.000000000000000000 ) ) ;
#109988=EDGE_CURVE ( 'NONE', #27877, #41297, #120212, .T. ) ;
#109989=ORIENTED_EDGE ( 'NONE', *, *, #110242, .F. ) ;
#109990=CARTESIAN_POINT ( 'NONE',  ( -6.900000000000019007, 2.500000000000000000, 0.4464101615137735513 ) ) ;
#109991=CARTESIAN_POINT ( 'NONE',  ( 7.899999999999923084, 12.50000000000000000, 0.6928203230275494784 ) ) ;
#109992=FACE_OUTER_BOUND ( 'NONE', #45556, .T. ) ;
#109993=ORIENTED_EDGE ( 'NONE', *, *, #61725, .T. ) ;
#109994=DIRECTION ( 'NONE',  ( -0.000000000000000000, 1.000000000000000000, -0.000000000000000000 ) ) ;
#109995=DIRECTION ( 'NONE',  ( 0.000000000000000000, 1.000000000000000000, 0.000000000000000000 ) ) ;
#109996=CARTESIAN_POINT ( 'NONE',  ( -11.44999999999999929, 2.500000000000000000, -6.148780366869522673 ) ) ;
#109997=EDGE_CURVE ( 'NONE', #73842, #59320, #19952, .T. ) ;
#109998=EDGE_CURVE ( 'NONE', #55268, #52643, #17788, .T. ) ;
#110000=LINE ( 'NONE', #67461, #84143 ) ;
#110001=EDGE_CURVE ( 'NONE', #126026, #17990, #99378, .T. ) ;
#110002=EDGE_CURVE ( 'NONE', #89736, #83886, #55457, .T. ) ;
#110003=CIRCLE ( 'NONE', #112151, 0.06509327318403745899 ) ;
#110004=DIRECTION ( 'NONE',  ( 0.000000000000000000, 0.000000000000000000, -1.000000000000000000 ) ) ;
#110005=EDGE_LOOP ( 'NONE', ( #115441, #72307 ) ) ;
#110006=ORIENTED_EDGE ( 'NONE', *, *, #49597, .F. ) ;
#110007=FACE_OUTER_BOUND ( 'NONE', #103726, .T. ) ;
#110008=EDGE_LOOP ( 'NONE', ( #15848, #109417 ) ) ;
#110009=CIRCLE ( 'NONE', #106081, 0.06509327318403745899 ) ;
#110010=FACE_OUTER_BOUND ( 'NONE', #114345, .T. ) ;
#110011=ORIENTED_EDGE ( 'NONE', *, *, #108993, .T. ) ;
#110012=ORIENTED_EDGE ( 'NONE', *, *, #124031, .F. ) ;
#110013=AXIS2_PLACEMENT_3D ( 'NONE', #69241, #50271, #71186 ) ;
#110014=VERTEX_POINT ( 'NONE', #123133 ) ;
#110015=EDGE_CURVE ( 'NONE', #106414, #27768, #13799, .T. ) ;
#110016=CARTESIAN_POINT ( 'NONE',  ( 87.50000000000000000, -1.433398978532513413, -7.395196794792769701 ) ) ;
#110017=CONICAL_SURFACE ( 'NONE', #101695, 0.1000000000000002554, 0.003490658503988666988 ) ;
#110018=ADVANCED_FACE ( 'NONE', ( #122492 ), #13675, .T. ) ;
#110019=FACE_OUTER_BOUND ( 'NONE', #116246, .T. ) ;
#110020=EDGE_CURVE ( 'NONE', #94676, #8586, #9485, .T. ) ;
#110021=FACE_OUTER_BOUND ( 'NONE', #5952, .T. ) ;
#110022=CIRCLE ( 'NONE', #13847, 0.06509327318403745899 ) ;
#110023=DIRECTION ( 'NONE',  ( 0.000000000000000000, -0.9999939076577903929, 0.003490651415223739937 ) ) ;
#110024=DIRECTION ( 'NONE',  ( -4.274815082592931898E-19, -0.9999939076577903929, -0.003490651415223739937 ) ) ;
#110025=CARTESIAN_POINT ( 'NONE',  ( 2.499999999999983569, 2.500000000000000000, -4.230127018922201998 ) ) ;
#110026=PLANE ( 'NONE',  #24660 ) ;
#110027=CARTESIAN_POINT ( 'NONE',  ( 9.349999999999919709, 2.500000000000000000, 2.511473670974873507 ) ) ;
#110028=PLANE ( 'NONE',  #106303 ) ;
#110029=VECTOR ( 'NONE', #29940, 1000.000000000000000 ) ;
#110030=ORIENTED_EDGE ( 'NONE', *, *, #5526, .T. ) ;
#110031=CIRCLE ( 'NONE', #124696, 0.06509327318403745899 ) ;
#110032=AXIS2_PLACEMENT_3D ( 'NONE', #63470, #62825, #52350 ) ;
#110034=EDGE_LOOP ( 'NONE', ( #120864, #78566, #64851, #110035 ) ) ;
#110035=ORIENTED_EDGE ( 'NONE', *, *, #1368, .F. ) ;
#110036=DIRECTION ( 'NONE',  ( 0.000000000000000000, -0.000000000000000000, 1.000000000000000000 ) ) ;
#110037=CARTESIAN_POINT ( 'NONE',  ( 5.599999999999931255, 2.500000000000000000, 3.983716857408420076 ) ) ;
#110039=CARTESIAN_POINT ( 'NONE',  ( 2.949999999999946887, 12.50000000000000000, -6.495190528383302464 ) ) ;
#110040=LINE ( 'NONE', #100215, #38602 ) ;
#110041=CARTESIAN_POINT ( 'NONE',  ( -1.250000000000036193, 2.500000000000000000, 1.572243186433545548 ) ) ;
#110042=ORIENTED_EDGE ( 'NONE', *, *, #100965, .F. ) ;
#110043=VERTEX_POINT ( 'NONE', #23634 ) ;
#110044=FACE_OUTER_BOUND ( 'NONE', #45401, .T. ) ;
#110045=VERTEX_POINT ( 'NONE', #92365 ) ;
#110047=ORIENTED_EDGE ( 'NONE', *, *, #18401, .F. ) ;
#110048=EDGE_CURVE ( 'NONE', #92609, #70125, #105636, .T. ) ;
#110049=ORIENTED_EDGE ( 'NONE', *, *, #90607, .F. ) ;
#110050=DIRECTION ( 'NONE',  ( 0.000000000000000000, -0.000000000000000000, 1.000000000000000000 ) ) ;
#110051=DIRECTION ( 'NONE',  ( 0.000000000000000000, 0.000000000000000000, -1.000000000000000000 ) ) ;
#110052=EDGE_CURVE ( 'NONE', #70966, #58229, #109835, .T. ) ;
#110053=AXIS2_PLACEMENT_3D ( 'NONE', #119814, #20331, #21619 ) ;
#110054=DIRECTION ( 'NONE',  ( 0.000000000000000000, -0.000000000000000000, 1.000000000000000000 ) ) ;
#110055=AXIS2_PLACEMENT_3D ( 'NONE', #113272, #125653, #84466 ) ;
#110056=FACE_OUTER_BOUND ( 'NONE', #11826, .T. ) ;
#110057=EDGE_CURVE ( 'NONE', #116464, #22615, #80512, .T. ) ;
#110058=CARTESIAN_POINT ( 'NONE',  ( -10.60000000000000142, 12.50000000000000000, 0.3464101615137736845 ) ) ;
#110059=ORIENTED_EDGE ( 'NONE', *, *, #70107, .T. ) ;
#110060=DIRECTION ( 'NONE',  ( -0.000000000000000000, 1.000000000000000000, -0.000000000000000000 ) ) ;
#110061=DIRECTION ( 'NONE',  ( 0.000000000000000000, 0.000000000000000000, -1.000000000000000000 ) ) ;
#110062=CARTESIAN_POINT ( 'NONE',  ( 1.849999999999950573, 12.50000000000000000, -1.753560074763288679 ) ) ;
#110063=DIRECTION ( 'NONE',  ( 0.000000000000000000, 0.000000000000000000, 1.000000000000000000 ) ) ;
#110064=EDGE_CURVE ( 'NONE', #114100, #89801, #42659, .T. ) ;
#110065=CIRCLE ( 'NONE', #107994, 0.1000000000000002554 ) ;
#110066=CIRCLE ( 'NONE', #11846, 0.06509327318403745899 ) ;
#110067=CARTESIAN_POINT ( 'NONE',  ( -2.300000000000033573, 2.500000000000000000, -3.983716857408426293 ) ) ;
#110068=VERTEX_POINT ( 'NONE', #81899 ) ;
#110069=ORIENTED_EDGE ( 'NONE', *, *, #84589, .F. ) ;
#110070=LINE ( 'NONE', #38777, #27850 ) ;
#110071=ORIENTED_EDGE ( 'NONE', *, *, #51081, .T. ) ;
#110072=CIRCLE ( 'NONE', #53631, 0.09999999999999982514 ) ;
#110073=DIRECTION ( 'NONE',  ( -0.000000000000000000, -1.000000000000000000, -0.000000000000000000 ) ) ;
#110074=DIRECTION ( 'NONE',  ( -0.000000000000000000, 1.000000000000000000, -0.000000000000000000 ) ) ;
#110075=CIRCLE ( 'NONE', #51597, 0.06509327318403745899 ) ;
#110076=ORIENTED_EDGE ( 'NONE', *, *, #105236, .F. ) ;
#110077=DIRECTION ( 'NONE',  ( -4.274815082592931898E-19, -0.9999939076577903929, -0.003490651415223739937 ) ) ;
#110078=FACE_OUTER_BOUND ( 'NONE', #40771, .T. ) ;
#110079=CARTESIAN_POINT ( 'NONE',  ( -2.050000000000032685, 12.50000000000000000, -2.099970236277064473 ) ) ;
#110080=EDGE_CURVE ( 'NONE', #91594, #30984, #24068, .T. ) ;
#110081=DIRECTION ( 'NONE',  ( 0.000000000000000000, 1.000000000000000000, 0.000000000000000000 ) ) ;
#110082=CARTESIAN_POINT ( 'NONE',  ( -10.45000000000000462, 2.500000000000000000, -2.065063509461098068 ) ) ;
#110083=ORIENTED_EDGE ( 'NONE', *, *, #23139, .F. ) ;
#110084=CARTESIAN_POINT ( 'NONE',  ( 59.88086527148990967, 3.776023839181152031, -4.996434403472031605 ) ) ;
#110085=CARTESIAN_POINT ( 'NONE',  ( 1.449999999999951772, 2.500000000000000000, -6.048780366869526581 ) ) ;
#110086=LINE ( 'NONE', #129111, #111896 ) ;
#110087=CIRCLE ( 'NONE', #3480, 0.06509327318403741736 ) ;
#110088=ORIENTED_EDGE ( 'NONE', *, *, #36245, .T. ) ;
#110089=CONICAL_SURFACE ( 'NONE', #36943, 0.1000000000000000472, 0.003490658503988666988 ) ;
#110090=EDGE_CURVE ( 'NONE', #104330, #27804, #76392, .T. ) ;
#110092=DIRECTION ( 'NONE',  ( -0.000000000000000000, -1.000000000000000000, -0.000000000000000000 ) ) ;
#110093=DIRECTION ( 'NONE',  ( 0.000000000000000000, 1.000000000000000000, 0.000000000000000000 ) ) ;
#110094=AXIS2_PLACEMENT_3D ( 'NONE', #93393, #73109, #34490 ) ;
#110096=AXIS2_PLACEMENT_3D ( 'NONE', #60084, #99998, #39165 ) ;
#110097=ORIENTED_EDGE ( 'NONE', *, *, #98631, .T. ) ;
#110098=DIRECTION ( 'NONE',  ( -0.000000000000000000, 1.000000000000000000, -0.000000000000000000 ) ) ;
#110099=CIRCLE ( 'NONE', #72556, 0.09999999999999982514 ) ;
#110100=CARTESIAN_POINT ( 'NONE',  ( -5.200000000000022382, 2.500000000000000000, 0.3464101615137735735 ) ) ;
#110101=VERTEX_POINT ( 'NONE', #82575 ) ;
#110102=CARTESIAN_POINT ( 'NONE',  ( -2.300000000000033573, 12.50000000000000000, 4.611443907251934426 ) ) ;
#110103=AXIS2_PLACEMENT_3D ( 'NONE', #113869, #24202, #6448 ) ;
#110104=EDGE_CURVE ( 'NONE', #48106, #11230, #82662, .T. ) ;
#110105=ORIENTED_EDGE ( 'NONE', *, *, #50618, .F. ) ;
#110106=DIRECTION ( 'NONE',  ( -4.274815082592931898E-19, -0.9999939076577903929, -0.003490651415223739937 ) ) ;
#110107=CIRCLE ( 'NONE', #101711, 0.1000000000000002554 ) ;
#110108=VECTOR ( 'NONE', #56066, 1000.000000000000000 ) ;
#110109=CIRCLE ( 'NONE', #108140, 0.1000000000000002554 ) ;
#110110=VERTEX_POINT ( 'NONE', #72745 ) ;
#110112=LINE ( 'NONE', #13829, #77251 ) ;
#110113=ORIENTED_EDGE ( 'NONE', *, *, #98876, .T. ) ;
#110114=EDGE_CURVE ( 'NONE', #56654, #37929, #53406, .T. ) ;
#110115=ORIENTED_EDGE ( 'NONE', *, *, #119772, .F. ) ;
#110116=CARTESIAN_POINT ( 'NONE',  ( 6.049999999999934097, 2.500000000000000000, -2.511473670974877948 ) ) ;
#110117=CARTESIAN_POINT ( 'NONE',  ( 4.399999999999937295, 2.500000000000000000, 3.883716857408421319 ) ) ;
#110118=VERTEX_POINT ( 'NONE', #62289 ) ;
#110119=CARTESIAN_POINT ( 'NONE',  ( -1.650000000000034772, 12.50000000000000000, 5.802370205355744659 ) ) ;
#110120=DIRECTION ( 'NONE',  ( 0.000000000000000000, -0.000000000000000000, 1.000000000000000000 ) ) ;
#110121=FACE_OUTER_BOUND ( 'NONE', #2529, .T. ) ;
#110122=CARTESIAN_POINT ( 'NONE',  ( 9.549999999999918998, 12.50000000000000000, 2.165063509461097713 ) ) ;
#110123=FACE_OUTER_BOUND ( 'NONE', #113824, .T. ) ;
#110124=LINE ( 'NONE', #2085, #53582 ) ;
#110125=DIRECTION ( 'NONE',  ( -0.000000000000000000, 1.000000000000000000, -0.000000000000000000 ) ) ;
#110126=AXIS2_PLACEMENT_3D ( 'NONE', #99374, #9694, #29351 ) ;
#110127=ORIENTED_EDGE ( 'NONE', *, *, #108201, .F. ) ;
#110128=EDGE_CURVE ( 'NONE', #61045, #4682, #102209, .T. ) ;
#110129=ORIENTED_EDGE ( 'NONE', *, *, #116176, .T. ) ;
#110130=ORIENTED_EDGE ( 'NONE', *, *, #63740, .F. ) ;
#110131=FACE_OUTER_BOUND ( 'NONE', #108870, .T. ) ;
#110132=DIRECTION ( 'NONE',  ( 0.000000000000000000, 0.000000000000000000, -1.000000000000000000 ) ) ;
#110133=CARTESIAN_POINT ( 'NONE',  ( 10.59999999999991260, 12.50000000000000000, 0.3464101615137735735 ) ) ;
#110134=VERTEX_POINT ( 'NONE', #43296 ) ;
#110135=VERTEX_POINT ( 'NONE', #112670 ) ;
#110136=FACE_BOUND ( 'NONE', #40968, .T. ) ;
#110137=EDGE_LOOP ( 'NONE', ( #80812, #13670, #74102, #2723 ) ) ;
#110138=CARTESIAN_POINT ( 'NONE',  ( -7.100000000000017408, 12.50000000000000000, -0.6928203230275542523 ) ) ;
#110139=DIRECTION ( 'NONE',  ( -0.000000000000000000, 1.000000000000000000, -0.000000000000000000 ) ) ;
#110140=CARTESIAN_POINT ( 'NONE',  ( 11.04999999999990656, 2.500000000000000000, -6.048780366869526581 ) ) ;
#110141=EDGE_CURVE ( 'NONE', #9133, #49498, #97217, .T. ) ;
#110142=FACE_OUTER_BOUND ( 'NONE', #108313, .T. ) ;
#110143=AXIS2_PLACEMENT_3D ( 'NONE', #40478, #79736, #119648 ) ;
#110144=DIRECTION ( 'NONE',  ( 0.000000000000000000, -0.000000000000000000, 1.000000000000000000 ) ) ;
#110145=CONICAL_SURFACE ( 'NONE', #53703, 0.1000000000000002554, 0.003490658503988666988 ) ;
#110146=DIRECTION ( 'NONE',  ( 0.000000000000000000, 0.000000000000000000, -1.000000000000000000 ) ) ;
#110147=LINE ( 'NONE', #109501, #35079 ) ;
#110148=DIRECTION ( 'NONE',  ( 0.000000000000000000, 1.000000000000000000, 0.000000000000000000 ) ) ;
#110149=EDGE_CURVE ( 'NONE', #105625, #83483, #55672, .T. ) ;
#110150=EDGE_CURVE ( 'NONE', #127039, #97686, #117056, .T. ) ;
#110151=CARTESIAN_POINT ( 'NONE',  ( -7.900000000000011013, 2.500000000000000000, 5.022947341949748790 ) ) ;
#110152=ADVANCED_FACE ( 'NONE', ( #115205 ), #45002, .T. ) ;
#110153=ADVANCED_FACE ( 'NONE', ( #85765 ), #5262, .T. ) ;
#110154=DIRECTION ( 'NONE',  ( 0.000000000000000000, 0.000000000000000000, -1.000000000000000000 ) ) ;
#110155=CIRCLE ( 'NONE', #24471, 0.1000000000000002554 ) ;
#110156=EDGE_LOOP ( 'NONE', ( #4476, #119128 ) ) ;
#110157=ORIENTED_EDGE ( 'NONE', *, *, #77205, .F. ) ;
#110158=ORIENTED_EDGE ( 'NONE', *, *, #96650, .T. ) ;
#110159=ORIENTED_EDGE ( 'NONE', *, *, #2436, .T. ) ;
#110160=DIRECTION ( 'NONE',  ( 0.000000000000000000, 0.000000000000000000, 1.000000000000000000 ) ) ;
#110161=EDGE_CURVE ( 'NONE', #112209, #85431, #61741, .T. ) ;
#110162=DIRECTION ( 'NONE',  ( 0.000000000000000000, 0.000000000000000000, -1.000000000000000000 ) ) ;
#110163=EDGE_CURVE ( 'NONE', #37879, #31124, #95168, .T. ) ;
#110164=ORIENTED_EDGE ( 'NONE', *, *, #79319, .F. ) ;
#110165=ORIENTED_EDGE ( 'NONE', *, *, #31437, .F. ) ;
#110166=ORIENTED_EDGE ( 'NONE', *, *, #63155, .F. ) ;
#110167=LINE ( 'NONE', #80061, #43840 ) ;
#110168=AXIS2_PLACEMENT_3D ( 'NONE', #129409, #55646, #37778 ) ;
#110169=CIRCLE ( 'NONE', #85014, 0.09999999999999999167 ) ;
#110170=EDGE_CURVE ( 'NONE', #112646, #101562, #67392, .T. ) ;
#110171=VECTOR ( 'NONE', #58474, 1000.000000000000000 ) ;
#110173=CARTESIAN_POINT ( 'NONE',  ( 7.499999999999961808, 12.50000000000000000, -4.330127018922201643 ) ) ;
#110174=DIRECTION ( 'NONE',  ( -0.000000000000000000, -1.000000000000000000, -0.000000000000000000 ) ) ;
#110175=DIRECTION ( 'NONE',  ( 0.000000000000000000, 0.000000000000000000, 1.000000000000000000 ) ) ;
#110176=PLANE ( 'NONE',  #24212 ) ;
#110177=CARTESIAN_POINT ( 'NONE',  ( 5.449999999999936229, 2.500000000000000000, 6.395190528383296602 ) ) ;
#110178=CARTESIAN_POINT ( 'NONE',  ( -0.8000000000000315747, 2.500000000000000000, 0.1000000000000000056 ) ) ;
#110179=ORIENTED_EDGE ( 'NONE', *, *, #1749, .T. ) ;
#110180=EDGE_CURVE ( 'NONE', #110134, #105827, #7201, .T. ) ;
#110181=DIRECTION ( 'NONE',  ( -0.000000000000000000, -1.000000000000000000, -0.000000000000000000 ) ) ;
#110182=ORIENTED_EDGE ( 'NONE', *, *, #36147, .F. ) ;
#110183=VERTEX_POINT ( 'NONE', #45221 ) ;
#110184=VERTEX_POINT ( 'NONE', #105427 ) ;
#110185=DIRECTION ( 'NONE',  ( -0.000000000000000000, 1.000000000000000000, -0.000000000000000000 ) ) ;
#110186=ORIENTED_EDGE ( 'NONE', *, *, #39520, .F. ) ;
#110187=AXIS2_PLACEMENT_3D ( 'NONE', #68446, #89392, #129339 ) ;
#110188=ORIENTED_EDGE ( 'NONE', *, *, #116064, .F. ) ;
#110189=AXIS2_PLACEMENT_3D ( 'NONE', #3415, #42728, #82635 ) ;
#110190=LINE ( 'NONE', #876, #84130 ) ;
#110191=DIRECTION ( 'NONE',  ( 0.000000000000000000, 0.000000000000000000, 1.000000000000000000 ) ) ;
#110192=AXIS2_PLACEMENT_3D ( 'NONE', #60537, #100434, #110886 ) ;
#110193=DIRECTION ( 'NONE',  ( -0.000000000000000000, -1.000000000000000000, -0.000000000000000000 ) ) ;
#110194=DIRECTION ( 'NONE',  ( -0.000000000000000000, 1.000000000000000000, -0.000000000000000000 ) ) ;
#110196=AXIS2_PLACEMENT_3D ( 'NONE', #10171, #100475, #50111 ) ;
#110197=CARTESIAN_POINT ( 'NONE',  ( 8.349999999999919709, 2.500000000000000000, 5.702370205355745014 ) ) ;
#110198=VECTOR ( 'NONE', #75043, 1000.000000000000000 ) ;
#110199=ORIENTED_EDGE ( 'NONE', *, *, #24921, .T. ) ;
#110200=CARTESIAN_POINT ( 'NONE',  ( 18.45986578164203351, 0.7763536479255011002, 4.045836815165626099 ) ) ;
#110201=ORIENTED_EDGE ( 'NONE', *, *, #4218, .F. ) ;
#110202=DIRECTION ( 'NONE',  ( 0.000000000000000000, 0.000000000000000000, 1.000000000000000000 ) ) ;
#110204=VERTEX_POINT ( 'NONE', #16997 ) ;
#110205=DIRECTION ( 'NONE',  ( 0.000000000000000000, 1.000000000000000000, 0.000000000000000000 ) ) ;
#110206=AXIS2_PLACEMENT_3D ( 'NONE', #76526, #84400, #124334 ) ;
#110207=DIRECTION ( 'NONE',  ( 0.000000000000000000, -0.9999939076577903929, 0.003490651415223739937 ) ) ;
#110208=EDGE_LOOP ( 'NONE', ( #122760, #54655 ) ) ;
#110209=ADVANCED_FACE ( 'NONE', ( #26223 ), #88998, .T. ) ;
#110210=AXIS2_PLACEMENT_3D ( 'NONE', #81526, #101814, #102455 ) ;
#110211=CIRCLE ( 'NONE', #22495, 0.09999999999999982514 ) ;
#110212=CARTESIAN_POINT ( 'NONE',  ( 4.149999999999941735, 12.50000000000000000, -7.122917578226816815 ) ) ;
#110213=EDGE_CURVE ( 'NONE', #89563, #107837, #56937, .T. ) ;
#110214=ORIENTED_EDGE ( 'NONE', *, *, #33764, .F. ) ;
#110215=VERTEX_POINT ( 'NONE', #125686 ) ;
#110216=DIRECTION ( 'NONE',  ( 0.000000000000000000, 1.000000000000000000, 0.000000000000000000 ) ) ;
#110217=CARTESIAN_POINT ( 'NONE',  ( 11.69999999999990870, 12.50000000000000000, -4.395220292106239768 ) ) ;
#110218=CARTESIAN_POINT ( 'NONE',  ( 4.549999999999939426, 12.50000000000000000, -6.495190528383302464 ) ) ;
#110219=CARTESIAN_POINT ( 'NONE',  ( 1.449999999999950440, 2.500000000000000000, 6.148780366869520009 ) ) ;
#110220=FACE_OUTER_BOUND ( 'NONE', #115334, .T. ) ;
#110221=ORIENTED_EDGE ( 'NONE', *, *, #129542, .T. ) ;
#110222=CARTESIAN_POINT ( 'NONE',  ( -7.499999999999976907, 12.50000000000000000, 4.265033745738159077 ) ) ;
#110223=CIRCLE ( 'NONE', #20341, 0.06509327318403745899 ) ;
#110224=ORIENTED_EDGE ( 'NONE', *, *, #76466, .T. ) ;
#110225=DIRECTION ( 'NONE',  ( 0.000000000000000000, -0.000000000000000000, 1.000000000000000000 ) ) ;
#110226=DIRECTION ( 'NONE',  ( -0.000000000000000000, -1.000000000000000000, -0.000000000000000000 ) ) ;
#110228=DIRECTION ( 'NONE',  ( 0.000000000000000000, -0.9999939076577903929, 0.003490651415223739937 ) ) ;
#110229=CARTESIAN_POINT ( 'NONE',  ( -1.250000000000001554, 2.500000000000000000, 2.165063509461097713 ) ) ;
#110232=ORIENTED_EDGE ( 'NONE', *, *, #64334, .T. ) ;
#110233=AXIS2_PLACEMENT_3D ( 'NONE', #119999, #78147, #119340 ) ;
#110234=CARTESIAN_POINT ( 'NONE',  ( 9.149999999999916866, 2.500000000000000000, -1.372243186433550033 ) ) ;
#110235=CONICAL_SURFACE ( 'NONE', #112390, 0.09999999999999982514, 0.003490658503988666988 ) ;
#110236=CARTESIAN_POINT ( 'NONE',  ( 11.44999999999990870, 2.500000000000000000, -1.818653347947326138 ) ) ;
#110237=DIRECTION ( 'NONE',  ( 0.000000000000000000, 1.000000000000000000, 0.000000000000000000 ) ) ;
#110238=EDGE_LOOP ( 'NONE', ( #24043, #123382, #109800, #89479 ) ) ;
#110239=VECTOR ( 'NONE', #2521, 1000.000000000000000 ) ;
#110240=AXIS2_PLACEMENT_3D ( 'NONE', #89617, #107969, #38605 ) ;
#110241=DIRECTION ( 'NONE',  ( 0.000000000000000000, 1.000000000000000000, 0.000000000000000000 ) ) ;
#110242=EDGE_CURVE ( 'NONE', #118390, #42458, #74328, .T. ) ;
#110243=AXIS2_PLACEMENT_3D ( 'NONE', #17083, #57703, #68144 ) ;
#110245=VERTEX_POINT ( 'NONE', #85126 ) ;
#110246=FACE_OUTER_BOUND ( 'NONE', #14931, .T. ) ;
#110247=VERTEX_POINT ( 'NONE', #75949 ) ;
#110248=DIRECTION ( 'NONE',  ( 0.000000000000000000, 0.000000000000000000, 1.000000000000000000 ) ) ;
#110249=FACE_OUTER_BOUND ( 'NONE', #91521, .T. ) ;
#110250=EDGE_LOOP ( 'NONE', ( #17842, #26265 ) ) ;
#110251=AXIS2_PLACEMENT_3D ( 'NONE', #100318, #51865, #70854 ) ;
#110252=CARTESIAN_POINT ( 'NONE',  ( -4.350000000000023626, 2.500000000000000000, 6.941600689897073018 ) ) ;
#110253=LINE ( 'NONE', #18642, #39022 ) ;
#110254=EDGE_CURVE ( 'NONE', #83521, #64553, #111990, .T. ) ;
#110255=CARTESIAN_POINT ( 'NONE',  ( -10.80000000000000071, 12.50000000000000000, -2.276824562219559311E-15 ) ) ;
#110256=EDGE_CURVE ( 'NONE', #27784, #103269, #55554, .T. ) ;
#110257=VERTEX_POINT ( 'NONE', #106066 ) ;
#110258=AXIS2_PLACEMENT_3D ( 'NONE', #65042, #95174, #123344 ) ;
#110259=EDGE_LOOP ( 'NONE', ( #95426, #59230, #51533, #63650 ) ) ;
#110260=ORIENTED_EDGE ( 'NONE', *, *, #78683, .F. ) ;
#110261=FACE_OUTER_BOUND ( 'NONE', #58955, .T. ) ;
#110262=DIRECTION ( 'NONE',  ( 0.000000000000000000, 1.000000000000000000, 0.000000000000000000 ) ) ;
#110263=CARTESIAN_POINT ( 'NONE',  ( 6.449999999999930012, 12.50000000000000000, 6.841600689897072485 ) ) ;
#110264=EDGE_CURVE ( 'NONE', #70439, #27091, #103674, .T. ) ;
#110265=FACE_BOUND ( 'NONE', #118830, .T. ) ;
#110266=ORIENTED_EDGE ( 'NONE', *, *, #77024, .T. ) ;
#110267=AXIS2_PLACEMENT_3D ( 'NONE', #56840, #7104, #115113 ) ;
#110268=DIRECTION ( 'NONE',  ( 0.000000000000000000, 1.000000000000000000, 0.000000000000000000 ) ) ;
#110269=LINE ( 'NONE', #40916, #85781 ) ;
#110270=VERTEX_POINT ( 'NONE', #96229 ) ;
#110272=DIRECTION ( 'NONE',  ( 0.000000000000000000, 1.000000000000000000, 0.000000000000000000 ) ) ;
#110274=DIRECTION ( 'NONE',  ( 0.000000000000000000, 0.000000000000000000, 1.000000000000000000 ) ) ;
#110275=CARTESIAN_POINT ( 'NONE',  ( 3.349999999999941913, 12.50000000000000000, 6.495190528383297135 ) ) ;
#110276=LINE ( 'NONE', #72301, #84316 ) ;
#110277=CARTESIAN_POINT ( 'NONE',  ( 10.39999999999991154, 2.500000000000000000, -4.922947341949753586 ) ) ;
#110278=AXIS2_PLACEMENT_3D ( 'NONE', #36263, #116095, #126570 ) ;
#110279=CARTESIAN_POINT ( 'NONE',  ( 1.849999999999949685, 2.500000000000000000, -2.511473670974877948 ) ) ;
#110280=CIRCLE ( 'NONE', #127016, 0.06509327318403745899 ) ;
#110281=AXIS2_PLACEMENT_3D ( 'NONE', #65435, #104086, #46437 ) ;
#110282=ORIENTED_EDGE ( 'NONE', *, *, #93955, .F. ) ;
#110283=ORIENTED_EDGE ( 'NONE', *, *, #51331, .T. ) ;
#110284=ORIENTED_EDGE ( 'NONE', *, *, #73148, .F. ) ;
#110285=VERTEX_POINT ( 'NONE', #6529 ) ;
#110286=DIRECTION ( 'NONE',  ( 0.000000000000000000, 0.000000000000000000, 1.000000000000000000 ) ) ;
#110287=CARTESIAN_POINT ( 'NONE',  ( 6.049999999999932321, 2.500000000000000000, -1.718653347947326049 ) ) ;
#110289=ORIENTED_EDGE ( 'NONE', *, *, #109079, .F. ) ;
#110290=FACE_BOUND ( 'NONE', #117399, .T. ) ;
#110291=CARTESIAN_POINT ( 'NONE',  ( 1.049999999999954969, 2.500000000000000000, -6.841600689897077814 ) ) ;
#110292=LINE ( 'NONE', #50728, #3102 ) ;
#110293=ADVANCED_FACE ( 'NONE', ( #126353 ), #20055, .T. ) ;
#110294=AXIS2_PLACEMENT_3D ( 'NONE', #121941, #42766, #32303 ) ;
#110295=VECTOR ( 'NONE', #68217, 1000.000000000000000 ) ;
#110296=DIRECTION ( 'NONE',  ( -0.000000000000000000, 1.000000000000000000, -0.000000000000000000 ) ) ;
#110297=CARTESIAN_POINT ( 'NONE',  ( 10.84999999999990905, 12.50000000000000000, -5.737276932171712751 ) ) ;
#110298=CARTESIAN_POINT ( 'NONE',  ( 9.999999999999952038, 2.500000000000000000, 0.09999999999999772959 ) ) ;
#110299=CARTESIAN_POINT ( 'NONE',  ( 8.949999999999921130, 2.500000000000000000, 1.718653347947321386 ) ) ;
#110300=CARTESIAN_POINT ( 'NONE',  ( 1.649999999999949729, 2.500000000000000000, 7.188010851410848723 ) ) ;
#110301=EDGE_CURVE ( 'NONE', #96482, #8842, #119110, .T. ) ;
#110302=DIRECTION ( 'NONE',  ( 0.000000000000000000, 1.000000000000000000, 0.000000000000000000 ) ) ;
#110303=ORIENTED_EDGE ( 'NONE', *, *, #15271, .F. ) ;
#110304=EDGE_CURVE ( 'NONE', #119380, #25933, #90941, .T. ) ;
#110305=ORIENTED_EDGE ( 'NONE', *, *, #3021, .T. ) ;
#110306=EDGE_LOOP ( 'NONE', ( #6431, #15898, #45621, #46552 ) ) ;
#110307=VERTEX_POINT ( 'NONE', #41218 ) ;
#110308=ORIENTED_EDGE ( 'NONE', *, *, #72742, .F. ) ;
#110309=ORIENTED_EDGE ( 'NONE', *, *, #87035, .F. ) ;
#110310=EDGE_CURVE ( 'NONE', #114671, #93896, #50366, .T. ) ;
#110311=LINE ( 'NONE', #41598, #90255 ) ;
#110312=EDGE_CURVE ( 'NONE', #75076, #104576, #119747, .T. ) ;
#110313=ADVANCED_FACE ( 'NONE', ( #109282 ), #60837, .T. ) ;
#110314=EDGE_LOOP ( 'NONE', ( #50436, #59329 ) ) ;
#110315=CIRCLE ( 'NONE', #53879, 0.06509327318403745899 ) ;
#110316=DIRECTION ( 'NONE',  ( -0.000000000000000000, 1.000000000000000000, -0.000000000000000000 ) ) ;
#110317=DIRECTION ( 'NONE',  ( -0.000000000000000000, -1.000000000000000000, -0.000000000000000000 ) ) ;
#110320=DIRECTION ( 'NONE',  ( 0.000000000000000000, 0.000000000000000000, 1.000000000000000000 ) ) ;
#110321=FACE_OUTER_BOUND ( 'NONE', #8745, .T. ) ;
#110322=EDGE_LOOP ( 'NONE', ( #53967, #71207 ) ) ;
#110323=FACE_OUTER_BOUND ( 'NONE', #46064, .T. ) ;
#110324=EDGE_CURVE ( 'NONE', #1853, #36682, #72283, .T. ) ;
#110325=AXIS2_PLACEMENT_3D ( 'NONE', #123842, #66215, #6620 ) ;
#110326=EDGE_LOOP ( 'NONE', ( #106094, #90457 ) ) ;
#110327=VECTOR ( 'NONE', #33465, 1000.000000000000000 ) ;
#110328=ORIENTED_EDGE ( 'NONE', *, *, #48962, .T. ) ;
#110329=DIRECTION ( 'NONE',  ( -0.000000000000000000, -1.000000000000000000, -0.000000000000000000 ) ) ;
#110330=LINE ( 'NONE', #71693, #124140 ) ;
#110331=DIRECTION ( 'NONE',  ( 0.000000000000000000, 0.000000000000000000, -1.000000000000000000 ) ) ;
#110332=ORIENTED_EDGE ( 'NONE', *, *, #126602, .T. ) ;
#110334=ORIENTED_EDGE ( 'NONE', *, *, #60059, .T. ) ;
#110335=CARTESIAN_POINT ( 'NONE',  ( 14.34999999999989662, 2.500000000000000000, 1.718653347947321386 ) ) ;
#110336=VECTOR ( 'NONE', #81978, 1000.000000000000000 ) ;
#110337=DIRECTION ( 'NONE',  ( 0.000000000000000000, 1.000000000000000000, 0.000000000000000000 ) ) ;
#110338=CARTESIAN_POINT ( 'NONE',  ( 10.59999999999990905, 12.50000000000000000, -3.983716857408426293 ) ) ;
#110339=DIRECTION ( 'NONE',  ( 0.000000000000000000, 0.000000000000000000, 1.000000000000000000 ) ) ;
#110340=EDGE_LOOP ( 'NONE', ( #107410, #887, #87745, #5962 ) ) ;
#110341=DIRECTION ( 'NONE',  ( 0.000000000000000000, 0.000000000000000000, -1.000000000000000000 ) ) ;
#110342=VERTEX_POINT ( 'NONE', #19623 ) ;
#110343=CARTESIAN_POINT ( 'NONE',  ( 7.049999999999926992, 12.50000000000000000, 2.165063509461097713 ) ) ;
#110344=ORIENTED_EDGE ( 'NONE', *, *, #112660, .T. ) ;
#110345=DIRECTION ( 'NONE',  ( 0.000000000000000000, 1.000000000000000000, 0.000000000000000000 ) ) ;
#110346=CARTESIAN_POINT ( 'NONE',  ( 1.449999999999952660, 12.50000000000000000, -6.841600689897078702 ) ) ;
#110347=DIRECTION ( 'NONE',  ( 0.000000000000000000, 1.000000000000000000, 0.000000000000000000 ) ) ;
#110348=AXIS2_PLACEMENT_3D ( 'NONE', #20547, #32963, #898 ) ;
#110349=DIRECTION ( 'NONE',  ( -4.274815082592931898E-19, -0.9999939076577903929, -0.003490651415223739937 ) ) ;
#110350=ORIENTED_EDGE ( 'NONE', *, *, #23081, .F. ) ;
#110351=CARTESIAN_POINT ( 'NONE',  ( -1.650000000000035216, 2.500000000000000000, -5.702370205355749455 ) ) ;
#110352=EDGE_CURVE ( 'NONE', #71169, #117955, #15826, .T. ) ;
#110353=CARTESIAN_POINT ( 'NONE',  ( 8.549999999999920774, 12.50000000000000000, 6.148780366869520897 ) ) ;
#110354=EDGE_LOOP ( 'NONE', ( #76195, #76004, #22901, #128354 ) ) ;
#110355=ORIENTED_EDGE ( 'NONE', *, *, #81961, .F. ) ;
#110356=ORIENTED_EDGE ( 'NONE', *, *, #51694, .F. ) ;
#110357=FACE_OUTER_BOUND ( 'NONE', #41624, .T. ) ;
#110358=CARTESIAN_POINT ( 'NONE',  ( 4.199999999999938005, 12.50000000000000000, 4.265033745738159077 ) ) ;
#110359=CARTESIAN_POINT ( 'NONE',  ( 18.70618316910014656, 2.558637580971261816, 2.503050677946378144 ) ) ;
#110360=LINE ( 'NONE', #1051, #14496 ) ;
#110361=DIRECTION ( 'NONE',  ( 0.000000000000000000, 0.000000000000000000, -1.000000000000000000 ) ) ;
#110362=AXIS2_PLACEMENT_3D ( 'NONE', #110649, #20982, #121114 ) ;
#110363=DIRECTION ( 'NONE',  ( -0.000000000000000000, -1.000000000000000000, -0.000000000000000000 ) ) ;
#110364=EDGE_CURVE ( 'NONE', #18875, #120364, #86929, .T. ) ;
#110365=AXIS2_PLACEMENT_3D ( 'NONE', #80795, #71599, #111524 ) ;
#110366=CARTESIAN_POINT ( 'NONE',  ( -3.749999999999991562, 2.500000000000000000, 6.495190528383297135 ) ) ;
#110367=DIRECTION ( 'NONE',  ( 0.000000000000000000, 1.000000000000000000, 0.000000000000000000 ) ) ;
#110369=AXIS2_PLACEMENT_3D ( 'NONE', #47363, #97102, #87270 ) ;
#110370=CIRCLE ( 'NONE', #36938, 0.1000000000000000472 ) ;
#110371=CONICAL_SURFACE ( 'NONE', #97764, 0.1000000000000002554, 0.003490658503988666988 ) ;
#110372=ORIENTED_EDGE ( 'NONE', *, *, #22584, .T. ) ;
#110373=CARTESIAN_POINT ( 'NONE',  ( 11.64999999999990266, 2.500000000000000000, -6.495190528383302464 ) ) ;
#110375=DIRECTION ( 'NONE',  ( -1.000000000000000000, -0.000000000000000000, -0.000000000000000000 ) ) ;
#110376=DIRECTION ( 'NONE',  ( 0.000000000000000000, 0.000000000000000000, 1.000000000000000000 ) ) ;
#110377=PLANE ( 'NONE',  #47969 ) ;
#110379=LINE ( 'NONE', #98607, #67543 ) ;
#110380=AXIS2_PLACEMENT_3D ( 'NONE', #124199, #44342, #42429 ) ;
#110381=AXIS2_PLACEMENT_3D ( 'NONE', #111348, #32830, #14439 ) ;
#110382=FACE_OUTER_BOUND ( 'NONE', #85409, .T. ) ;
#110383=FACE_OUTER_BOUND ( 'NONE', #52494, .T. ) ;
#110384=ORIENTED_EDGE ( 'NONE', *, *, #27680, .F. ) ;
#110385=ORIENTED_EDGE ( 'NONE', *, *, #53673, .T. ) ;
#110386=DIRECTION ( 'NONE',  ( 0.000000000000000000, 0.000000000000000000, 1.000000000000000000 ) ) ;
#110387=EDGE_CURVE ( 'NONE', #46747, #48610, #63957, .T. ) ;
#110388=ORIENTED_EDGE ( 'NONE', *, *, #20352, .F. ) ;
#110389=ORIENTED_EDGE ( 'NONE', *, *, #117350, .T. ) ;
#110390=LINE ( 'NONE', #71768, #128206 ) ;
#110391=DIRECTION ( 'NONE',  ( 0.000000000000000000, 0.000000000000000000, -1.000000000000000000 ) ) ;
#110393=DIRECTION ( 'NONE',  ( -0.000000000000000000, 1.000000000000000000, -0.000000000000000000 ) ) ;
#110394=EDGE_CURVE ( 'NONE', #112569, #71600, #107775, .T. ) ;
#110395=ORIENTED_EDGE ( 'NONE', *, *, #85496, .T. ) ;
#110396=VECTOR ( 'NONE', #102728, 1000.000000000000000 ) ;
#110397=AXIS2_PLACEMENT_3D ( 'NONE', #15650, #5830, #45789 ) ;
#110398=DIRECTION ( 'NONE',  ( 0.000000000000000000, 0.000000000000000000, 1.000000000000000000 ) ) ;
#110399=ORIENTED_EDGE ( 'NONE', *, *, #108839, .F. ) ;
#110400=DIRECTION ( 'NONE',  ( -0.000000000000000000, -1.000000000000000000, -0.000000000000000000 ) ) ;
#110401=CIRCLE ( 'NONE', #26791, 0.1000000000000002554 ) ;
#110402=EDGE_CURVE ( 'NONE', #54998, #117091, #80597, .T. ) ;
#110403=CARTESIAN_POINT ( 'NONE',  ( 17.49999999999999645, 2.500000000000056843, 3.093179327514578691 ) ) ;
#110404=CARTESIAN_POINT ( 'NONE',  ( -5.400000000000020783, 2.500000000000000000, 5.022947341949748790 ) ) ;
#110405=EDGE_CURVE ( 'NONE', #94349, #107710, #128299, .T. ) ;
#110406=ORIENTED_EDGE ( 'NONE', *, *, #110264, .T. ) ;
#110407=CONICAL_SURFACE ( 'NONE', #58104, 0.1000000000000002554, 0.003490658503988666988 ) ;
#110408=AXIS2_PLACEMENT_3D ( 'NONE', #53523, #113730, #24059 ) ;
#110409=ORIENTED_EDGE ( 'NONE', *, *, #20146, .F. ) ;
#110410=ADVANCED_FACE ( 'NONE', ( #70651 ), #10440, .T. ) ;
#110411=ORIENTED_EDGE ( 'NONE', *, *, #81741, .T. ) ;
#110412=VERTEX_POINT ( 'NONE', #79201 ) ;
#110413=ORIENTED_EDGE ( 'NONE', *, *, #102583, .T. ) ;
#110414=DIRECTION ( 'NONE',  ( 0.000000000000000000, -0.9999939076577903929, 0.003490651415223739937 ) ) ;
#110415=CARTESIAN_POINT ( 'NONE',  ( 9.112263991918691630, 2.499999999999745537, 9.392448312006688838 ) ) ;
#110416=DIRECTION ( 'NONE',  ( 0.000000000000000000, -0.000000000000000000, 1.000000000000000000 ) ) ;
#110417=EDGE_CURVE ( 'NONE', #86684, #102251, #126657, .T. ) ;
#110418=FACE_BOUND ( 'NONE', #105231, .T. ) ;
#110419=CARTESIAN_POINT ( 'NONE',  ( -12.69999999999999396, 12.50000000000000000, 0.3464101615137776813 ) ) ;
#110421=AXIS2_PLACEMENT_3D ( 'NONE', #123602, #36544, #33955 ) ;
#110422=CARTESIAN_POINT ( 'NONE',  ( 12.29999999999990479, 12.50000000000000000, -3.983716857408426293 ) ) ;
#110423=DIRECTION ( 'NONE',  ( 0.000000000000000000, 0.000000000000000000, 1.000000000000000000 ) ) ;
#110424=AXIS2_PLACEMENT_3D ( 'NONE', #12994, #33325, #3212 ) ;
#110425=CARTESIAN_POINT ( 'NONE',  ( -2.700000000000029932, 2.500000000000000000, -0.3464101615137782364 ) ) ;
#110426=FACE_OUTER_BOUND ( 'NONE', #94376, .T. ) ;
#110427=DIRECTION ( 'NONE',  ( 0.000000000000000000, 0.000000000000000000, 1.000000000000000000 ) ) ;
#110428=AXIS2_PLACEMENT_3D ( 'NONE', #96129, #118347, #6426 ) ;
#110429=DIRECTION ( 'NONE',  ( 0.000000000000000000, 0.000000000000000000, 1.000000000000000000 ) ) ;
#110431=ORIENTED_EDGE ( 'NONE', *, *, #63749, .F. ) ;
#110432=ORIENTED_EDGE ( 'NONE', *, *, #3334, .F. ) ;
#110433=VERTEX_POINT ( 'NONE', #129602 ) ;
#110434=AXIS2_PLACEMENT_3D ( 'NONE', #83956, #54500, #15861 ) ;
#110435=PLANE ( 'NONE',  #114979 ) ;
#110436=CARTESIAN_POINT ( 'NONE',  ( 5.599999999999933031, 2.500000000000000000, -0.3464101615137783474 ) ) ;
#110437=FACE_BOUND ( 'NONE', #49793, .T. ) ;
#110438=CARTESIAN_POINT ( 'NONE',  ( -9.150000000000009237, 2.500000000000000000, -2.165063509461101710 ) ) ;
#110439=AXIS2_PLACEMENT_3D ( 'NONE', #124860, #44356, #4403 ) ;
#110440=EDGE_CURVE ( 'NONE', #26624, #123305, #1163, .T. ) ;
#110442=ORIENTED_EDGE ( 'NONE', *, *, #78978, .T. ) ;
#110443=DIRECTION ( 'NONE',  ( 0.000000000000000000, 0.000000000000000000, 1.000000000000000000 ) ) ;
#110444=DIRECTION ( 'NONE',  ( 0.000000000000000000, 1.000000000000000000, 0.000000000000000000 ) ) ;
#110446=DIRECTION ( 'NONE',  ( 0.000000000000000000, 0.000000000000000000, -1.000000000000000000 ) ) ;
#110447=VERTEX_POINT ( 'NONE', #109945 ) ;
#110449=CARTESIAN_POINT ( 'NONE',  ( -11.84999999999999609, 12.50000000000000000, 1.818653347947321475 ) ) ;
#110450=ADVANCED_FACE ( 'NONE', ( #90270 ), #612, .T. ) ;
#110451=CIRCLE ( 'NONE', #114653, 0.06509327318403745899 ) ;
#110452=ORIENTED_EDGE ( 'NONE', *, *, #44552, .T. ) ;
#110453=ORIENTED_EDGE ( 'NONE', *, *, #36687, .F. ) ;
#110454=ADVANCED_FACE ( 'NONE', ( #72598 ), #23483, .T. ) ;
#110455=CARTESIAN_POINT ( 'NONE',  ( 5.599999999999931255, 12.50000000000000000, 4.676537180435972552 ) ) ;
#110457=CIRCLE ( 'NONE', #47777, 0.06509327318403741736 ) ;
#110458=EDGE_CURVE ( 'NONE', #8336, #22036, #76485, .T. ) ;
#110459=VERTEX_POINT ( 'NONE', #101411 ) ;
#110460=DIRECTION ( 'NONE',  ( -0.000000000000000000, -1.000000000000000000, -0.000000000000000000 ) ) ;
#110461=ADVANCED_FACE ( 'NONE', ( #31391 ), #118240, .T. ) ;
#110462=CARTESIAN_POINT ( 'NONE',  ( -3.300000000000028244, 2.500000000000000000, 4.330127018922196314 ) ) ;
#110463=DIRECTION ( 'NONE',  ( 0.000000000000000000, 0.000000000000000000, -1.000000000000000000 ) ) ;
#110464=DIRECTION ( 'NONE',  ( 0.000000000000000000, 1.000000000000000000, 0.000000000000000000 ) ) ;
#110465=EDGE_CURVE ( 'NONE', #21250, #55865, #30531, .T. ) ;
#110466=VERTEX_POINT ( 'NONE', #64057 ) ;
#110467=AXIS2_PLACEMENT_3D ( 'NONE', #43657, #104487, #92750 ) ;
#110468=FACE_OUTER_BOUND ( 'NONE', #62052, .T. ) ;
#110469=ORIENTED_EDGE ( 'NONE', *, *, #103214, .F. ) ;
#110470=FACE_OUTER_BOUND ( 'NONE', #76932, .T. ) ;
#110471=ADVANCED_FACE ( 'NONE', ( #43795 ), #32589, .T. ) ;
#110472=AXIS2_PLACEMENT_3D ( 'NONE', #94500, #82780, #73567 ) ;
#110473=CONICAL_SURFACE ( 'NONE', #87478, 0.09999999999999999167, 0.003490658503988666988 ) ;
#110474=ADVANCED_FACE ( 'NONE', ( #11731 ), #84788, .T. ) ;
#110475=EDGE_LOOP ( 'NONE', ( #3029, #20975 ) ) ;
#110476=DIRECTION ( 'NONE',  ( -0.000000000000000000, 1.000000000000000000, -0.000000000000000000 ) ) ;
#110477=ORIENTED_EDGE ( 'NONE', *, *, #53586, .F. ) ;
#110478=FACE_OUTER_BOUND ( 'NONE', #5675, .T. ) ;
#110479=DIRECTION ( 'NONE',  ( -0.000000000000000000, 1.000000000000000000, -0.000000000000000000 ) ) ;
#110480=CARTESIAN_POINT ( 'NONE',  ( -11.64999999999999680, 2.500000000000000000, -7.188010851410850499 ) ) ;
#110481=DIRECTION ( 'NONE',  ( 0.000000000000000000, 1.000000000000000000, 0.000000000000000000 ) ) ;
#110482=DIRECTION ( 'NONE',  ( 0.000000000000000000, 0.000000000000000000, 1.000000000000000000 ) ) ;
#110483=ORIENTED_EDGE ( 'NONE', *, *, #117217, .T. ) ;
#110484=ORIENTED_EDGE ( 'NONE', *, *, #113129, .F. ) ;
#110485=EDGE_LOOP ( 'NONE', ( #108060, #27811 ) ) ;
#110486=DIRECTION ( 'NONE',  ( 0.000000000000000000, 0.000000000000000000, 1.000000000000000000 ) ) ;
#110487=DIRECTION ( 'NONE',  ( 0.000000000000000000, 0.000000000000000000, -1.000000000000000000 ) ) ;
#110488=FACE_OUTER_BOUND ( 'NONE', #35084, .T. ) ;
#110489=AXIS2_PLACEMENT_3D ( 'NONE', #40612, #21581, #61525 ) ;
#110491=ORIENTED_EDGE ( 'NONE', *, *, #170, .T. ) ;
#110492=ORIENTED_EDGE ( 'NONE', *, *, #94052, .F. ) ;
#110493=CARTESIAN_POINT ( 'NONE',  ( -10.65000000000000213, 12.50000000000000000, 1.818653347947321475 ) ) ;
#110494=ORIENTED_EDGE ( 'NONE', *, *, #20669, .F. ) ;
#110495=FACE_OUTER_BOUND ( 'NONE', #49791, .T. ) ;
#110496=AXIS2_PLACEMENT_3D ( 'NONE', #62263, #31500, #41341 ) ;
#110497=CIRCLE ( 'NONE', #108431, 0.1000000000000002554 ) ;
#110498=FACE_OUTER_BOUND ( 'NONE', #83806, .T. ) ;
#110499=CARTESIAN_POINT ( 'NONE',  ( -14.59999999999998366, 12.50000000000000000, -0.06509327318403752838 ) ) ;
#110500=CIRCLE ( 'NONE', #31102, 0.06509327318403745899 ) ;
#110501=LINE ( 'NONE', #79126, #115434 ) ;
#110502=CARTESIAN_POINT ( 'NONE',  ( -12.09999999999999609, 2.500000000000000000, -3.537306695894647302 ) ) ;
#110503=CARTESIAN_POINT ( 'NONE',  ( -1.450000000000035483, 2.500000000000000000, 1.818653347947321475 ) ) ;
#110504=PLANE ( 'NONE',  #20721 ) ;
#110505=CONICAL_SURFACE ( 'NONE', #125081, 0.1000000000000002554, 0.003490658503988666988 ) ;
#110506=ORIENTED_EDGE ( 'NONE', *, *, #50606, .T. ) ;
#110507=VECTOR ( 'NONE', #38733, 1000.000000000000000 ) ;
#110508=VERTEX_POINT ( 'NONE', #4457 ) ;
#110509=CONICAL_SURFACE ( 'NONE', #95929, 0.09999999999999982514, 0.003490658503988666988 ) ;
#110510=CARTESIAN_POINT ( 'NONE',  ( -12.09999999999999609, 12.50000000000000000, 0.6277270498435161272 ) ) ;
#110511=AXIS2_PLACEMENT_3D ( 'NONE', #12575, #62349, #173 ) ;
#110512=CARTESIAN_POINT ( 'NONE',  ( 13.09999999999990195, 12.50000000000000000, -3.983716857408426293 ) ) ;
#110513=EDGE_LOOP ( 'NONE', ( #32156, #14280, #2054, #62718 ) ) ;
#110514=VERTEX_POINT ( 'NONE', #53604 ) ;
#110516=CARTESIAN_POINT ( 'NONE',  ( 13.14999999999989733, 12.50000000000000000, -2.511473670974877948 ) ) ;
#110518=DIRECTION ( 'NONE',  ( 0.000000000000000000, -0.9999939076577903929, 0.003490651415223739937 ) ) ;
#110519=DIRECTION ( 'NONE',  ( 0.000000000000000000, 0.000000000000000000, -1.000000000000000000 ) ) ;
#110520=EDGE_CURVE ( 'NONE', #12748, #19409, #33958, .T. ) ;
#110521=CIRCLE ( 'NONE', #129329, 0.1000000000000002554 ) ;
#110522=DIRECTION ( 'NONE',  ( 0.000000000000000000, -0.9999939076577903929, 0.003490651415223739937 ) ) ;
#110523=DIRECTION ( 'NONE',  ( 0.000000000000000000, -0.9999939076577903929, 0.003490651415223739937 ) ) ;
#110524=CARTESIAN_POINT ( 'NONE',  ( -0.4000000000000339950, 12.50000000000000000, 0.6928203230275518099 ) ) ;
#110525=PLANE ( 'NONE',  #8174 ) ;
#110526=CONICAL_SURFACE ( 'NONE', #120994, 0.1000000000000000056, 0.003490658503988666988 ) ;
#110527=ORIENTED_EDGE ( 'NONE', *, *, #118236, .T. ) ;
#110528=EDGE_LOOP ( 'NONE', ( #15851, #84012, #17949, #76321 ) ) ;
#110529=ORIENTED_EDGE ( 'NONE', *, *, #3901, .T. ) ;
#110530=CONICAL_SURFACE ( 'NONE', #102222, 0.09999999999999982514, 0.003490658503988666988 ) ;
#110531=ORIENTED_EDGE ( 'NONE', *, *, #120792, .F. ) ;
#110532=EDGE_LOOP ( 'NONE', ( #87916, #105500, #37858, #18076 ) ) ;
#110533=DIRECTION ( 'NONE',  ( 0.000000000000000000, 0.000000000000000000, 1.000000000000000000 ) ) ;
#110534=DIRECTION ( 'NONE',  ( 0.000000000000000000, -0.000000000000000000, 1.000000000000000000 ) ) ;
#110536=FACE_OUTER_BOUND ( 'NONE', #60072, .T. ) ;
#110537=CARTESIAN_POINT ( 'NONE',  ( -7.500000000000015099, 2.500000000000000000, -0.7928203230275542301 ) ) ;
#110538=AXIS2_PLACEMENT_3D ( 'NONE', #29870, #69793, #107783 ) ;
#110539=CARTESIAN_POINT ( 'NONE',  ( 4.149999999999941735, 12.50000000000000000, -2.857883832488653741 ) ) ;
#110540=DIRECTION ( 'NONE',  ( 0.000000000000000000, -0.9999939076577903929, 0.003490651415223739937 ) ) ;
#110541=ORIENTED_EDGE ( 'NONE', *, *, #78736, .F. ) ;
#110542=LINE ( 'NONE', #60177, #9789 ) ;
#110543=AXIS2_PLACEMENT_3D ( 'NONE', #45483, #85388, #99085 ) ;
#110544=DIRECTION ( 'NONE',  ( -0.000000000000000000, 1.000000000000000000, -0.000000000000000000 ) ) ;
#110545=EDGE_LOOP ( 'NONE', ( #85912, #101848 ) ) ;
#110546=AXIS2_PLACEMENT_3D ( 'NONE', #26855, #127629, #107339 ) ;
#110547=ORIENTED_EDGE ( 'NONE', *, *, #44817, .F. ) ;
#110548=EDGE_LOOP ( 'NONE', ( #103068, #122476, #64422, #90475 ) ) ;
#110549=ORIENTED_EDGE ( 'NONE', *, *, #76937, .F. ) ;
#110550=CARTESIAN_POINT ( 'NONE',  ( -4.200000000000025935, 2.500000000000000000, 4.330127018922196314 ) ) ;
#110551=CONICAL_SURFACE ( 'NONE', #100099, 0.1000000000000002554, 0.003490658503988666988 ) ;
#110552=DIRECTION ( 'NONE',  ( 0.000000000000000000, 0.000000000000000000, 1.000000000000000000 ) ) ;
#110553=DIRECTION ( 'NONE',  ( -0.000000000000000000, -1.000000000000000000, -0.000000000000000000 ) ) ;
#110554=ADVANCED_FACE ( 'NONE', ( #61496 ), #5362, .T. ) ;
#110555=AXIS2_PLACEMENT_3D ( 'NONE', #61616, #75755, #72711 ) ;
#110556=AXIS2_PLACEMENT_3D ( 'NONE', #615, #11733, #109286 ) ;
#110557=PLANE ( 'NONE',  #55 ) ;
#110558=EDGE_LOOP ( 'NONE', ( #64532, #40127 ) ) ;
#110559=DIRECTION ( 'NONE',  ( 0.000000000000000000, 1.000000000000000000, 0.000000000000000000 ) ) ;
#110560=DIRECTION ( 'NONE',  ( 0.000000000000000000, 0.000000000000000000, 1.000000000000000000 ) ) ;
#110561=EDGE_CURVE ( 'NONE', #85675, #89168, #61819, .T. ) ;
#110562=DIRECTION ( 'NONE',  ( 0.000000000000000000, -0.9999939076577903929, 0.003490651415223739937 ) ) ;
#110563=CARTESIAN_POINT ( 'NONE',  ( 10.59999999999991260, 2.500000000000000000, -0.2464101615137783419 ) ) ;
#110564=EDGE_CURVE ( 'NONE', #113036, #43893, #99473, .T. ) ;
#110565=ORIENTED_EDGE ( 'NONE', *, *, #105090, .F. ) ;
#110566=AXIS2_PLACEMENT_3D ( 'NONE', #44347, #15523, #124206 ) ;
#110567=CIRCLE ( 'NONE', #33321, 0.06509327318403745899 ) ;
#110568=ORIENTED_EDGE ( 'NONE', *, *, #90036, .F. ) ;
#110569=EDGE_CURVE ( 'NONE', #30363, #51458, #70314, .T. ) ;
#110570=ADVANCED_FACE ( 'NONE', ( #71284 ), #82429, .T. ) ;
#110571=ORIENTED_EDGE ( 'NONE', *, *, #44976, .T. ) ;
#110572=CARTESIAN_POINT ( 'NONE',  ( 7.899999999999921307, 2.500000000000000000, 0.09999999999999761857 ) ) ;
#110573=ADVANCED_FACE ( 'NONE', ( #62140 ), #45186, .T. ) ;
#110574=CARTESIAN_POINT ( 'NONE',  ( -3.950000000000026379, 2.500000000000000000, -1.818653347947326138 ) ) ;
#110575=EDGE_CURVE ( 'NONE', #127721, #95822, #80693, .T. ) ;
#110576=FACE_BOUND ( 'NONE', #101734, .T. ) ;
#110577=DIRECTION ( 'NONE',  ( -0.000000000000000000, 1.000000000000000000, -0.000000000000000000 ) ) ;
#110578=DIRECTION ( 'NONE',  ( 0.000000000000000000, 0.000000000000000000, -1.000000000000000000 ) ) ;
#110579=DIRECTION ( 'NONE',  ( 0.000000000000000000, -0.000000000000000000, 1.000000000000000000 ) ) ;
#110580=CONICAL_SURFACE ( 'NONE', #8166, 0.09999999999999982514, 0.003490658503988666988 ) ;
#110581=CARTESIAN_POINT ( 'NONE',  ( 8.349999999999919709, 2.500000000000000000, -2.857883832488653741 ) ) ;
#110582=CARTESIAN_POINT ( 'NONE',  ( -6.450000000000014388, 2.500000000000000000, 1.718653347947321386 ) ) ;
#110583=DIRECTION ( 'NONE',  ( 0.000000000000000000, 0.000000000000000000, 1.000000000000000000 ) ) ;
#110584=EDGE_LOOP ( 'NONE', ( #105518, #2643, #112139, #3740 ) ) ;
#110585=DIRECTION ( 'NONE',  ( -0.000000000000000000, -1.000000000000000000, -0.000000000000000000 ) ) ;
#110586=AXIS2_PLACEMENT_3D ( 'NONE', #58874, #28129, #30074 ) ;
#110587=AXIS2_PLACEMENT_3D ( 'NONE', #58227, #77204, #99436 ) ;
#110588=LINE ( 'NONE', #100750, #64181 ) ;
#110589=ORIENTED_EDGE ( 'NONE', *, *, #94180, .F. ) ;
#110590=EDGE_LOOP ( 'NONE', ( #96907, #115739 ) ) ;
#110592=FACE_OUTER_BOUND ( 'NONE', #23772, .T. ) ;
#110593=FACE_BOUND ( 'NONE', #99312, .T. ) ;
#110594=CARTESIAN_POINT ( 'NONE',  ( 0.8499999999999553468, 2.500000000000000000, 1.572243186433545548 ) ) ;
#110595=AXIS2_PLACEMENT_3D ( 'NONE', #109872, #30681, #42426 ) ;
#110596=CIRCLE ( 'NONE', #116843, 0.06509327318403745899 ) ;
#110597=FACE_OUTER_BOUND ( 'NONE', #24845, .T. ) ;
#110598=VERTEX_POINT ( 'NONE', #102054 ) ;
#110599=DIRECTION ( 'NONE',  ( 0.000000000000000000, 0.000000000000000000, 1.000000000000000000 ) ) ;
#110600=EDGE_CURVE ( 'NONE', #73675, #81499, #32694, .T. ) ;
#110602=CIRCLE ( 'NONE', #20728, 0.09999999999999982514 ) ;
#110603=ORIENTED_EDGE ( 'NONE', *, *, #97307, .F. ) ;
#110604=CARTESIAN_POINT ( 'NONE',  ( 5.849999999999932143, 12.50000000000000000, 1.472243186433545459 ) ) ;
#110605=DIRECTION ( 'NONE',  ( -0.000000000000000000, -1.000000000000000000, -0.000000000000000000 ) ) ;
#110606=CONICAL_SURFACE ( 'NONE', #83438, 0.1000000000000002554, 0.003490658503988666988 ) ;
#110607=EDGE_CURVE ( 'NONE', #89861, #6770, #105814, .T. ) ;
#110608=EDGE_CURVE ( 'NONE', #55865, #14057, #65984, .T. ) ;
#110609=CARTESIAN_POINT ( 'NONE',  ( -4.400000000000028777, 12.50000000000000000, -4.676537180435978769 ) ) ;
#110611=ADVANCED_FACE ( 'NONE', ( #15584 ), #87025, .T. ) ;
#110612=ORIENTED_EDGE ( 'NONE', *, *, #103502, .T. ) ;
#110613=CARTESIAN_POINT ( 'NONE',  ( -5.400000000000023448, 12.50000000000000000, -4.395220292106239768 ) ) ;
#110614=DIRECTION ( 'NONE',  ( 0.000000000000000000, 1.000000000000000000, 0.000000000000000000 ) ) ;
#110615=DIRECTION ( 'NONE',  ( -0.000000000000000000, 1.000000000000000000, -0.000000000000000000 ) ) ;
#110616=AXIS2_PLACEMENT_3D ( 'NONE', #99061, #8711, #61054 ) ;
#110617=EDGE_CURVE ( 'NONE', #38921, #86526, #84977, .T. ) ;
#110618=ORIENTED_EDGE ( 'NONE', *, *, #126373, .F. ) ;
#110619=VERTEX_POINT ( 'NONE', #126851 ) ;
#110620=EDGE_CURVE ( 'NONE', #92178, #29080, #53594, .T. ) ;
#110622=EDGE_CURVE ( 'NONE', #67678, #98580, #1261, .T. ) ;
#110623=ORIENTED_EDGE ( 'NONE', *, *, #82137, .F. ) ;
#110624=FACE_OUTER_BOUND ( 'NONE', #124944, .T. ) ;
#110625=DIRECTION ( 'NONE',  ( 0.000000000000000000, 0.000000000000000000, 1.000000000000000000 ) ) ;
#110626=EDGE_CURVE ( 'NONE', #96049, #72066, #40996, .T. ) ;
#110627=EDGE_CURVE ( 'NONE', #124289, #91471, #114123, .T. ) ;
#110628=CARTESIAN_POINT ( 'NONE',  ( 9.149999999999916866, 12.50000000000000000, 5.802370205355744659 ) ) ;
#110629=ORIENTED_EDGE ( 'NONE', *, *, #113353, .T. ) ;
#110630=DIRECTION ( 'NONE',  ( 0.000000000000000000, 0.000000000000000000, -1.000000000000000000 ) ) ;
#110631=DIRECTION ( 'NONE',  ( 0.000000000000000000, 1.000000000000000000, 0.000000000000000000 ) ) ;
#110632=DIRECTION ( 'NONE',  ( 0.000000000000000000, 0.000000000000000000, -1.000000000000000000 ) ) ;
#110634=DIRECTION ( 'NONE',  ( 0.000000000000000000, 0.000000000000000000, 1.000000000000000000 ) ) ;
#110635=DIRECTION ( 'NONE',  ( 0.000000000000000000, 1.000000000000000000, 0.000000000000000000 ) ) ;
#110636=EDGE_CURVE ( 'NONE', #95428, #65807, #95454, .T. ) ;
#110637=EDGE_LOOP ( 'NONE', ( #19935, #18848 ) ) ;
#110638=ORIENTED_EDGE ( 'NONE', *, *, #17757, .F. ) ;
#110639=CARTESIAN_POINT ( 'NONE',  ( -12.94999999999999218, 12.50000000000000000, -2.099970236277062252 ) ) ;
#110640=ORIENTED_EDGE ( 'NONE', *, *, #100537, .T. ) ;
#110642=VERTEX_POINT ( 'NONE', #107192 ) ;
#110643=EDGE_LOOP ( 'NONE', ( #127615, #51944, #61546, #63468 ) ) ;
#110644=ORIENTED_EDGE ( 'NONE', *, *, #69607, .F. ) ;
#110645=AXIS2_PLACEMENT_3D ( 'NONE', #89874, #100355, #29674 ) ;
#110646=CARTESIAN_POINT ( 'NONE',  ( 17.50000000000000000, -0.8333333333333287074, -3.999999999999996447 ) ) ;
#110647=EDGE_CURVE ( 'NONE', #112093, #25877, #77102, .T. ) ;
#110648=PLANE ( 'NONE',  #27648 ) ;
#110649=CARTESIAN_POINT ( 'NONE',  ( 5.849999999999934808, 12.50000000000000000, -5.802370205355749988 ) ) ;
#110650=VECTOR ( 'NONE', #41706, 1000.000000000000000 ) ;
#110651=CARTESIAN_POINT ( 'NONE',  ( 10.64999999999990976, 12.50000000000000000, 2.511473670974873507 ) ) ;
#110652=DIRECTION ( 'NONE',  ( -0.000000000000000000, 1.000000000000000000, -0.000000000000000000 ) ) ;
#110653=FACE_OUTER_BOUND ( 'NONE', #83458, .T. ) ;
#110654=DIRECTION ( 'NONE',  ( 0.000000000000000000, 0.000000000000000000, -1.000000000000000000 ) ) ;
#110655=CARTESIAN_POINT ( 'NONE',  ( -14.14999999999998792, 12.50000000000000000, 2.792790559304615616 ) ) ;
#110656=CIRCLE ( 'NONE', #127391, 0.1000000000000002554 ) ;
#110657=CARTESIAN_POINT ( 'NONE',  ( 4.999999999999935163, 2.500000000000000000, 3.637306695894644726 ) ) ;
#110658=AXIS2_PLACEMENT_3D ( 'NONE', #116832, #126009, #36374 ) ;
#110659=EDGE_LOOP ( 'NONE', ( #51627, #67938, #108978, #2047 ) ) ;
#110660=CARTESIAN_POINT ( 'NONE',  ( 11.64999999999990266, 2.500000000000000000, 2.065063509461097624 ) ) ;
#110661=ORIENTED_EDGE ( 'NONE', *, *, #45852, .F. ) ;
#110662=ORIENTED_EDGE ( 'NONE', *, *, #39245, .T. ) ;
#110663=DIRECTION ( 'NONE',  ( 0.000000000000000000, 0.000000000000000000, -1.000000000000000000 ) ) ;
#110664=CARTESIAN_POINT ( 'NONE',  ( 11.64999999999990798, 2.500000000000000000, 7.288010851410849256 ) ) ;
#110666=EDGE_CURVE ( 'NONE', #60337, #17483, #74425, .T. ) ;
#110667=CARTESIAN_POINT ( 'NONE',  ( 2.499999999999983569, 12.50000000000000000, -4.330127018922201643 ) ) ;
#110668=FACE_OUTER_BOUND ( 'NONE', #81294, .T. ) ;
#110669=DIRECTION ( 'NONE',  ( 0.000000000000000000, 1.000000000000000000, 0.000000000000000000 ) ) ;
#110670=CONICAL_SURFACE ( 'NONE', #8259, 0.1000000000000000472, 0.003490658503988666988 ) ;
#110671=ORIENTED_EDGE ( 'NONE', *, *, #66472, .T. ) ;
#110672=ORIENTED_EDGE ( 'NONE', *, *, #33794, .F. ) ;
#110673=AXIS2_PLACEMENT_3D ( 'NONE', #75764, #65293, #64027 ) ;
#110674=FACE_OUTER_BOUND ( 'NONE', #95121, .T. ) ;
#110675=VERTEX_POINT ( 'NONE', #64695 ) ;
#110676=CARTESIAN_POINT ( 'NONE',  ( -13.14999999999999147, 12.50000000000000000, -1.818653347947323917 ) ) ;
#110677=ORIENTED_EDGE ( 'NONE', *, *, #33389, .F. ) ;
#110678=EDGE_CURVE ( 'NONE', #99586, #98405, #82848, .T. ) ;
#110679=VERTEX_POINT ( 'NONE', #6385 ) ;
#110680=CARTESIAN_POINT ( 'NONE',  ( 13.74999999999989875, 2.500000000000000000, 1.372243186433545370 ) ) ;
#110681=CONICAL_SURFACE ( 'NONE', #29139, 0.1000000000000002554, 0.003490658503988666988 ) ;
#110682=DIRECTION ( 'NONE',  ( -0.000000000000000000, -1.000000000000000000, -0.000000000000000000 ) ) ;
#110683=CONICAL_SURFACE ( 'NONE', #64716, 0.1000000000000002554, 0.003490658503988666988 ) ;
#110684=CARTESIAN_POINT ( 'NONE',  ( 5.399999999999933742, 12.50000000000000000, 0.06509327318403504425 ) ) ;
#110685=CARTESIAN_POINT ( 'NONE',  ( -7.700000000000010836, 2.500000000000000000, 3.883716857408421319 ) ) ;
#110686=DIRECTION ( 'NONE',  ( 0.000000000000000000, 0.000000000000000000, 1.000000000000000000 ) ) ;
#110687=EDGE_LOOP ( 'NONE', ( #89604, #47756 ) ) ;
#110688=CARTESIAN_POINT ( 'NONE',  ( -3.550000000000028688, 2.500000000000000000, 6.841600689897072485 ) ) ;
#110689=DIRECTION ( 'NONE',  ( 0.000000000000000000, 0.000000000000000000, -1.000000000000000000 ) ) ;
#110690=DIRECTION ( 'NONE',  ( 0.000000000000000000, -0.9999939076577903929, 0.003490651415223739937 ) ) ;
#110691=CARTESIAN_POINT ( 'NONE',  ( -8.100000000000013856, 12.50000000000000000, 0.3464101615137736845 ) ) ;
#110692=AXIS2_PLACEMENT_3D ( 'NONE', #32862, #62314, #12540 ) ;
#110693=CARTESIAN_POINT ( 'NONE',  ( -5.000000000000023093, 2.500000000000000000, 5.122947341949749323 ) ) ;
#110694=CIRCLE ( 'NONE', #39630, 0.09999999999999982514 ) ;
#110695=EDGE_LOOP ( 'NONE', ( #128214, #12590, #68149, #62915 ) ) ;
#110696=VECTOR ( 'NONE', #34929, 1000.000000000000000 ) ;
#110697=ORIENTED_EDGE ( 'NONE', *, *, #106319, .F. ) ;
#110699=VERTEX_POINT ( 'NONE', #75169 ) ;
#110700=CARTESIAN_POINT ( 'NONE',  ( 6.649999999999931077, 2.500000000000000000, -6.395190528383301931 ) ) ;
#110701=DIRECTION ( 'NONE',  ( 0.000000000000000000, 0.000000000000000000, -1.000000000000000000 ) ) ;
#110702=EDGE_CURVE ( 'NONE', #36641, #38962, #103764, .T. ) ;
#110703=AXIS2_PLACEMENT_3D ( 'NONE', #73448, #102284, #4687 ) ;
#110704=VERTEX_POINT ( 'NONE', #25397 ) ;
#110706=DIRECTION ( 'NONE',  ( 0.000000000000000000, 1.000000000000000000, 0.000000000000000000 ) ) ;
#110707=CARTESIAN_POINT ( 'NONE',  ( 2.499999999999981792, 2.500000000000000000, 4.230127018922196669 ) ) ;
#110708=PLANE ( 'NONE',  #116574 ) ;
#110709=EDGE_CURVE ( 'NONE', #91784, #126895, #65328, .T. ) ;
#110710=DIRECTION ( 'NONE',  ( -0.000000000000000000, -1.000000000000000000, -0.000000000000000000 ) ) ;
#110711=ORIENTED_EDGE ( 'NONE', *, *, #60626, .T. ) ;
#110712=EDGE_CURVE ( 'NONE', #32237, #5152, #126751, .T. ) ;
#110713=EDGE_CURVE ( 'NONE', #12498, #114933, #26073, .T. ) ;
#110714=ADVANCED_FACE ( 'NONE', ( #56154 ), #17977, .T. ) ;
#110715=CARTESIAN_POINT ( 'NONE',  ( 76.45228544977298668, 3.905198701529716487, -5.870122411652127781 ) ) ;
#110716=EDGE_CURVE ( 'NONE', #73698, #110699, #51454, .T. ) ;
#110718=CARTESIAN_POINT ( 'NONE',  ( -7.300000000000018474, 2.500000000000000000, -3.883716857408426648 ) ) ;
#110719=CARTESIAN_POINT ( 'NONE',  ( 1.249999999999950262, 12.50000000000000000, 7.188010851410848723 ) ) ;
#110720=DIRECTION ( 'NONE',  ( -4.274815082592931898E-19, -0.9999939076577903929, -0.003490651415223739937 ) ) ;
#110721=ORIENTED_EDGE ( 'NONE', *, *, #44054, .F. ) ;
#110723=CARTESIAN_POINT ( 'NONE',  ( 11.64999999999990266, 2.500000000000000000, -6.595190528383302109 ) ) ;
#110724=VECTOR ( 'NONE', #79742, 1000.000000000000000 ) ;
#110725=CARTESIAN_POINT ( 'NONE',  ( -3.550000000000028688, 12.50000000000000000, 6.906693963081109722 ) ) ;
#110726=ADVANCED_FACE ( 'NONE', ( #128138 ), #10293, .T. ) ;
#110727=CARTESIAN_POINT ( 'NONE',  ( 9.349999999999919709, 2.500000000000000000, -6.841600689897078702 ) ) ;
#110728=EDGE_LOOP ( 'NONE', ( #42351, #126293 ) ) ;
#110729=EDGE_CURVE ( 'NONE', #86633, #63267, #120255, .T. ) ;
#110730=CARTESIAN_POINT ( 'NONE',  ( 7.499999999999961808, 2.500000000000000000, 4.330127018922196314 ) ) ;
#110731=EDGE_CURVE ( 'NONE', #118967, #40079, #84878, .T. ) ;
#110732=AXIS2_PLACEMENT_3D ( 'NONE', #25871, #63864, #103137 ) ;
#110734=DIRECTION ( 'NONE',  ( -0.000000000000000000, -1.000000000000000000, -0.000000000000000000 ) ) ;
#110735=VECTOR ( 'NONE', #85342, 1000.000000000000000 ) ;
#110736=VERTEX_POINT ( 'NONE', #60061 ) ;
#110737=LINE ( 'NONE', #11243, #9225 ) ;
#110738=ORIENTED_EDGE ( 'NONE', *, *, #81302, .T. ) ;
#110739=CARTESIAN_POINT ( 'NONE',  ( -3.550000000000027356, 12.50000000000000000, -2.511473670974877948 ) ) ;
#110740=AXIS2_PLACEMENT_3D ( 'NONE', #46620, #86545, #107482 ) ;
#110741=AXIS2_PLACEMENT_3D ( 'NONE', #64200, #5275, #33476 ) ;
#110742=VERTEX_POINT ( 'NONE', #9646 ) ;
#110743=DIRECTION ( 'NONE',  ( -0.000000000000000000, 1.000000000000000000, -0.000000000000000000 ) ) ;
#110744=FACE_OUTER_BOUND ( 'NONE', #91166, .T. ) ;
#110745=ORIENTED_EDGE ( 'NONE', *, *, #39063, .F. ) ;
#110746=ORIENTED_EDGE ( 'NONE', *, *, #82734, .T. ) ;
#110747=DIRECTION ( 'NONE',  ( -0.000000000000000000, 1.000000000000000000, -0.000000000000000000 ) ) ;
#110748=CARTESIAN_POINT ( 'NONE',  ( -4.600000000000024514, 12.50000000000000000, 5.022947341949748790 ) ) ;
#110749=VERTEX_POINT ( 'NONE', #10900 ) ;
#110750=DIRECTION ( 'NONE',  ( -0.000000000000000000, -1.000000000000000000, -0.000000000000000000 ) ) ;
#110752=CARTESIAN_POINT ( 'NONE',  ( -8.150000000000014566, 2.500000000000000000, -6.148780366869520897 ) ) ;
#110753=DIRECTION ( 'NONE',  ( 0.000000000000000000, 1.000000000000000000, 0.000000000000000000 ) ) ;
#110754=DIRECTION ( 'NONE',  ( 0.000000000000000000, 0.000000000000000000, 1.000000000000000000 ) ) ;
#110755=DIRECTION ( 'NONE',  ( -0.000000000000000000, 1.000000000000000000, -0.000000000000000000 ) ) ;
#110756=DIRECTION ( 'NONE',  ( -0.000000000000000000, -1.000000000000000000, -0.000000000000000000 ) ) ;
#110757=CONICAL_SURFACE ( 'NONE', #41748, 0.1000000000000000472, 0.003490658503988666988 ) ;
#110758=VECTOR ( 'NONE', #6134, 1000.000000000000000 ) ;
#110759=ORIENTED_EDGE ( 'NONE', *, *, #86774, .T. ) ;
#110760=ORIENTED_EDGE ( 'NONE', *, *, #2090, .F. ) ;
#110761=DIRECTION ( 'NONE',  ( 0.000000000000000000, 0.000000000000000000, -1.000000000000000000 ) ) ;
#110762=VERTEX_POINT ( 'NONE', #99966 ) ;
#110763=DIRECTION ( 'NONE',  ( -0.000000000000000000, -1.000000000000000000, -0.000000000000000000 ) ) ;
#110764=DIRECTION ( 'NONE',  ( -0.000000000000000000, 1.000000000000000000, -0.000000000000000000 ) ) ;
#110765=LINE ( 'NONE', #2096, #69966 ) ;
#110766=ORIENTED_EDGE ( 'NONE', *, *, #68521, .T. ) ;
#110767=VERTEX_POINT ( 'NONE', #37817 ) ;
#110768=FACE_BOUND ( 'NONE', #12433, .T. ) ;
#110769=ORIENTED_EDGE ( 'NONE', *, *, #72402, .T. ) ;
#110770=ADVANCED_FACE ( 'NONE', ( #30595 ), #32684, .T. ) ;
#110771=DIRECTION ( 'NONE',  ( 0.000000000000000000, 0.000000000000000000, 1.000000000000000000 ) ) ;
#110772=CARTESIAN_POINT ( 'NONE',  ( -7.700000000000016165, 12.50000000000000000, 0.3464101615137735735 ) ) ;
#110773=CONICAL_SURFACE ( 'NONE', #102381, 0.09999999999999982514, 0.003490658503988666988 ) ;
#110774=EDGE_CURVE ( 'NONE', #12584, #49114, #99570, .T. ) ;
#110775=CARTESIAN_POINT ( 'NONE',  ( -9.800000000000004263, 2.500000000000000000, -0.2464101615137783419 ) ) ;
#110776=CARTESIAN_POINT ( 'NONE',  ( 1.449999999999951772, 2.500000000000000000, -6.148780366869526226 ) ) ;
#110777=LINE ( 'NONE', #80696, #122377 ) ;
#110778=EDGE_CURVE ( 'NONE', #88035, #87323, #59875, .T. ) ;
#110779=DIRECTION ( 'NONE',  ( 0.000000000000000000, 0.000000000000000000, -1.000000000000000000 ) ) ;
#110780=DIRECTION ( 'NONE',  ( 0.000000000000000000, 0.000000000000000000, -1.000000000000000000 ) ) ;
#110781=DIRECTION ( 'NONE',  ( -0.000000000000000000, 1.000000000000000000, -0.000000000000000000 ) ) ;
#110782=LINE ( 'NONE', #121900, #24503 ) ;
#110783=CARTESIAN_POINT ( 'NONE',  ( 0.5999999999999560130, 2.500000000000000000, -3.983716857408426293 ) ) ;
#110784=CIRCLE ( 'NONE', #12579, 0.06509327318403745899 ) ;
#110785=CARTESIAN_POINT ( 'NONE',  ( 11.44999999999990692, 12.50000000000000000, 1.753560074763284016 ) ) ;
#110786=EDGE_CURVE ( 'NONE', #47422, #124116, #20136, .T. ) ;
#110787=AXIS2_PLACEMENT_3D ( 'NONE', #26365, #47939, #97668 ) ;
#110788=ORIENTED_EDGE ( 'NONE', *, *, #88736, .T. ) ;
#110789=VERTEX_POINT ( 'NONE', #39141 ) ;
#110790=AXIS2_PLACEMENT_3D ( 'NONE', #100275, #62295, #90428 ) ;
#110791=VERTEX_POINT ( 'NONE', #70495 ) ;
#110792=ORIENTED_EDGE ( 'NONE', *, *, #104997, .T. ) ;
#110793=CARTESIAN_POINT ( 'NONE',  ( 7.499999999999927169, 2.500000000000000000, 3.637306695894644726 ) ) ;
#110794=DIRECTION ( 'NONE',  ( 0.000000000000000000, 0.000000000000000000, -1.000000000000000000 ) ) ;
#110795=EDGE_LOOP ( 'NONE', ( #106825, #50052 ) ) ;
#110796=VERTEX_POINT ( 'NONE', #90117 ) ;
#110797=AXIS2_PLACEMENT_3D ( 'NONE', #97589, #67459, #47865 ) ;
#110798=VERTEX_POINT ( 'NONE', #129453 ) ;
#110799=CARTESIAN_POINT ( 'NONE',  ( 3.099999999999944134, 12.50000000000000000, 4.676537180435972552 ) ) ;
#110800=DIRECTION ( 'NONE',  ( -0.000000000000000000, -1.000000000000000000, -0.000000000000000000 ) ) ;
#110802=LINE ( 'NONE', #112108, #50123 ) ;
#110803=DIRECTION ( 'NONE',  ( -0.000000000000000000, 1.000000000000000000, -0.000000000000000000 ) ) ;
#110804=DIRECTION ( 'NONE',  ( -0.000000000000000000, 1.000000000000000000, -0.000000000000000000 ) ) ;
#110805=CARTESIAN_POINT ( 'NONE',  ( 0.3999999999999568345, 12.50000000000000000, -5.022947341949754119 ) ) ;
#110806=EDGE_CURVE ( 'NONE', #20024, #84209, #36866, .T. ) ;
#110807=VERTEX_POINT ( 'NONE', #80330 ) ;
#110808=CARTESIAN_POINT ( 'NONE',  ( -8.749999999999975131, 12.50000000000000000, 2.165063509461097713 ) ) ;
#110809=ORIENTED_EDGE ( 'NONE', *, *, #23443, .F. ) ;
#110810=VERTEX_POINT ( 'NONE', #79049 ) ;
#110811=ORIENTED_EDGE ( 'NONE', *, *, #25160, .F. ) ;
#110812=CARTESIAN_POINT ( 'NONE',  ( -1.450000000000035483, 2.500000000000000000, 1.718653347947321386 ) ) ;
#110813=ORIENTED_EDGE ( 'NONE', *, *, #18075, .F. ) ;
#110814=VERTEX_POINT ( 'NONE', #20755 ) ;
#110815=ORIENTED_EDGE ( 'NONE', *, *, #112367, .F. ) ;
#110816=DIRECTION ( 'NONE',  ( 0.000000000000000000, 0.000000000000000000, 1.000000000000000000 ) ) ;
#110817=CARTESIAN_POINT ( 'NONE',  ( -1.900000000000034106, 2.500000000000000000, -3.983716857408426293 ) ) ;
#110818=CARTESIAN_POINT ( 'NONE',  ( -8.350000000000012079, 2.500000000000000000, -2.857883832488653741 ) ) ;
#110819=EDGE_CURVE ( 'NONE', #115252, #90867, #118952, .T. ) ;
#110820=DIRECTION ( 'NONE',  ( 0.000000000000000000, 0.000000000000000000, 1.000000000000000000 ) ) ;
#110821=CARTESIAN_POINT ( 'NONE',  ( 6.649999999999929301, 2.500000000000000000, -2.065063509461102065 ) ) ;
#110822=AXIS2_PLACEMENT_3D ( 'NONE', #61248, #40327, #112286 ) ;
#110823=LINE ( 'NONE', #61091, #21170 ) ;
#110824=CARTESIAN_POINT ( 'NONE',  ( -10.85000000000000142, 2.500000000000000000, -2.165063509461097713 ) ) ;
#110825=ORIENTED_EDGE ( 'NONE', *, *, #79699, .F. ) ;
#110826=DIRECTION ( 'NONE',  ( 0.000000000000000000, 0.000000000000000000, -1.000000000000000000 ) ) ;
#110827=CIRCLE ( 'NONE', #54392, 0.1000000000000002554 ) ;
#110828=CIRCLE ( 'NONE', #54393, 0.06509327318403745899 ) ;
#110829=ORIENTED_EDGE ( 'NONE', *, *, #69188, .F. ) ;
#110830=CARTESIAN_POINT ( 'NONE',  ( 1.249999999999986899, 12.50000000000000000, 6.430097255199259010 ) ) ;
#110831=DIRECTION ( 'NONE',  ( -4.274815082592931898E-19, -0.9999939076577903929, -0.003490651415223739937 ) ) ;
#110832=EDGE_LOOP ( 'NONE', ( #111867, #52040, #75506, #11700 ) ) ;
#110833=DIRECTION ( 'NONE',  ( 0.000000000000000000, -0.000000000000000000, 1.000000000000000000 ) ) ;
#110834=ADVANCED_FACE ( 'NONE', ( #127496 ), #8347, .T. ) ;
#110835=LINE ( 'NONE', #120672, #39521 ) ;
#110836=ORIENTED_EDGE ( 'NONE', *, *, #71297, .T. ) ;
#110837=AXIS2_PLACEMENT_3D ( 'NONE', #115681, #53073, #16179 ) ;
#110838=CARTESIAN_POINT ( 'NONE',  ( -1.700000000000034817, 12.50000000000000000, -2.385244779468109755E-15 ) ) ;
#110839=EDGE_LOOP ( 'NONE', ( #59207, #66243, #58520, #53372 ) ) ;
#110840=VERTEX_POINT ( 'NONE', #98653 ) ;
#110842=DIRECTION ( 'NONE',  ( 0.000000000000000000, 1.000000000000000000, 0.000000000000000000 ) ) ;
#110843=DIRECTION ( 'NONE',  ( -4.274815082592931898E-19, -0.9999939076577903929, -0.003490651415223739937 ) ) ;
#110844=DIRECTION ( 'NONE',  ( 0.000000000000000000, -0.9999939076577903929, 0.003490651415223739937 ) ) ;
#110845=DIRECTION ( 'NONE',  ( -4.274815082592931898E-19, -0.9999939076577903929, -0.003490651415223739937 ) ) ;
#110847=DIRECTION ( 'NONE',  ( -0.000000000000000000, 1.000000000000000000, -0.000000000000000000 ) ) ;
#110848=EDGE_LOOP ( 'NONE', ( #38845, #5826 ) ) ;
#110849=DIRECTION ( 'NONE',  ( 0.000000000000000000, 1.000000000000000000, 0.000000000000000000 ) ) ;
#110850=CONICAL_SURFACE ( 'NONE', #46036, 0.1000000000000002554, 0.003490658503988666988 ) ;
#110851=DIRECTION ( 'NONE',  ( 0.000000000000000000, 0.000000000000000000, 1.000000000000000000 ) ) ;
#110852=CIRCLE ( 'NONE', #96265, 0.1000000000000000056 ) ;
#110853=EDGE_CURVE ( 'NONE', #120047, #4792, #27999, .T. ) ;
#110855=DIRECTION ( 'NONE',  ( -0.000000000000000000, 1.000000000000000000, -0.000000000000000000 ) ) ;
#110856=FACE_OUTER_BOUND ( 'NONE', #128999, .T. ) ;
#110857=DIRECTION ( 'NONE',  ( 0.000000000000000000, 0.000000000000000000, 1.000000000000000000 ) ) ;
#110858=CARTESIAN_POINT ( 'NONE',  ( 4.599999999999940137, 12.50000000000000000, -4.957854068765716882 ) ) ;
#110859=ORIENTED_EDGE ( 'NONE', *, *, #83225, .F. ) ;
#110860=CIRCLE ( 'NONE', #117112, 0.1000000000000002554 ) ;
#110861=EDGE_CURVE ( 'NONE', #51834, #117332, #64047, .T. ) ;
#110862=DIRECTION ( 'NONE',  ( 0.000000000000000000, 0.000000000000000000, -1.000000000000000000 ) ) ;
#110863=LINE ( 'NONE', #21206, #85130 ) ;
#110864=EDGE_CURVE ( 'NONE', #45163, #35141, #95353, .T. ) ;
#110865=EDGE_CURVE ( 'NONE', #124496, #4260, #64134, .T. ) ;
#110866=EDGE_CURVE ( 'NONE', #129005, #88166, #87113, .T. ) ;
#110867=EDGE_CURVE ( 'NONE', #128878, #107859, #103854, .T. ) ;
#110868=ORIENTED_EDGE ( 'NONE', *, *, #5515, .T. ) ;
#110869=LINE ( 'NONE', #101064, #107503 ) ;
#110870=CIRCLE ( 'NONE', #83707, 0.1000000000000000472 ) ;
#110871=CIRCLE ( 'NONE', #69017, 0.09999999999999982514 ) ;
#110872=VERTEX_POINT ( 'NONE', #120882 ) ;
#110873=ORIENTED_EDGE ( 'NONE', *, *, #120967, .T. ) ;
#110874=CARTESIAN_POINT ( 'NONE',  ( -3.550000000000027356, 2.500000000000000000, 1.818653347947321475 ) ) ;
#110875=EDGE_CURVE ( 'NONE', #43219, #72747, #16003, .T. ) ;
#110876=EDGE_CURVE ( 'NONE', #22096, #80261, #57793, .T. ) ;
#110877=VERTEX_POINT ( 'NONE', #34938 ) ;
#110878=DIRECTION ( 'NONE',  ( 0.000000000000000000, 0.000000000000000000, 1.000000000000000000 ) ) ;
#110879=CARTESIAN_POINT ( 'NONE',  ( -3.350000000000028511, 2.500000000000000000, -1.472243186433550122 ) ) ;
#110880=CARTESIAN_POINT ( 'NONE',  ( 12.89999999999990266, 2.500000000000000000, 3.637306695894644726 ) ) ;
#110881=ADVANCED_FACE ( 'NONE', ( #114758 ), #7686, .T. ) ;
#110882=ORIENTED_EDGE ( 'NONE', *, *, #71243, .F. ) ;
#110883=EDGE_CURVE ( 'NONE', #74144, #1435, #34295, .T. ) ;
#110884=CARTESIAN_POINT ( 'NONE',  ( -0.8500000000000382805, 12.50000000000000000, -2.857883832488653741 ) ) ;
#110885=ADVANCED_FACE ( 'NONE', ( #114122 ), #105906, .T. ) ;
#110886=DIRECTION ( 'NONE',  ( 0.000000000000000000, 0.000000000000000000, -1.000000000000000000 ) ) ;
#110887=CIRCLE ( 'NONE', #73327, 0.1000000000000002554 ) ;
#110888=DIRECTION ( 'NONE',  ( 0.000000000000000000, 0.000000000000000000, -1.000000000000000000 ) ) ;
#110889=EDGE_CURVE ( 'NONE', #10941, #29719, #128920, .T. ) ;
#110890=ORIENTED_EDGE ( 'NONE', *, *, #40031, .T. ) ;
#110891=ORIENTED_EDGE ( 'NONE', *, *, #57832, .T. ) ;
#110892=VERTEX_POINT ( 'NONE', #74851 ) ;
#110893=CARTESIAN_POINT ( 'NONE',  ( -7.499999999999980460, 2.500000000000000000, -2.276824562219559311E-15 ) ) ;
#110894=CARTESIAN_POINT ( 'NONE',  ( -5.200000000000020606, 12.50000000000000000, -0.4115034346978156399 ) ) ;
#110895=LINE ( 'NONE', #120727, #27521 ) ;
#110896=FACE_BOUND ( 'NONE', #50935, .T. ) ;
#110897=ORIENTED_EDGE ( 'NONE', *, *, #43099, .T. ) ;
#110898=PLANE ( 'NONE',  #111827 ) ;
#110899=CARTESIAN_POINT ( 'NONE',  ( 5.849999999999933920, 2.500000000000000000, 6.395190528383296602 ) ) ;
#110900=ORIENTED_EDGE ( 'NONE', *, *, #113838, .T. ) ;
#110901=DIRECTION ( 'NONE',  ( -0.000000000000000000, -1.000000000000000000, -0.000000000000000000 ) ) ;
#110902=DIRECTION ( 'NONE',  ( 0.000000000000000000, -0.000000000000000000, 1.000000000000000000 ) ) ;
#110903=CONICAL_SURFACE ( 'NONE', #52425, 0.1000000000000000472, 0.003490658503988666988 ) ;
#110904=DIRECTION ( 'NONE',  ( 0.000000000000000000, 0.000000000000000000, 1.000000000000000000 ) ) ;
#110905=CARTESIAN_POINT ( 'NONE',  ( -8.100000000000013856, 2.500000000000000000, -4.083716857408426826 ) ) ;
#110906=CARTESIAN_POINT ( 'NONE',  ( -5.000000000000023093, 2.500000000000000000, 5.022947341949748790 ) ) ;
#110907=AXIS2_PLACEMENT_3D ( 'NONE', #53860, #16484, #75416 ) ;
#110908=AXIS2_PLACEMENT_3D ( 'NONE', #111634, #31785, #42252 ) ;
#110909=CARTESIAN_POINT ( 'NONE',  ( -10.00000000000000533, 2.500000000000000000, 0.6928203230275494784 ) ) ;
#110910=LINE ( 'NONE', #22566, #50442 ) ;
#110911=AXIS2_PLACEMENT_3D ( 'NONE', #98967, #59050, #60968 ) ;
#110912=VERTEX_POINT ( 'NONE', #80970 ) ;
#110913=ORIENTED_EDGE ( 'NONE', *, *, #103657, .F. ) ;
#110914=ORIENTED_EDGE ( 'NONE', *, *, #111580, .F. ) ;
#110915=EDGE_LOOP ( 'NONE', ( #70826, #39054, #54175, #82493 ) ) ;
#110916=CARTESIAN_POINT ( 'NONE',  ( -12.49999999999999467, 2.500000000000000000, 0.6928203230275535862 ) ) ;
#110917=LINE ( 'NONE', #21254, #4912 ) ;
#110918=ORIENTED_EDGE ( 'NONE', *, *, #121126, .T. ) ;
#110919=FACE_BOUND ( 'NONE', #22752, .T. ) ;
#110920=LINE ( 'NONE', #59286, #98040 ) ;
#110921=ADVANCED_FACE ( 'NONE', ( #105606 ), #65001, .T. ) ;
#110922=DIRECTION ( 'NONE',  ( 0.000000000000000000, 1.000000000000000000, 0.000000000000000000 ) ) ;
#110923=CARTESIAN_POINT ( 'NONE',  ( -4.150000000000028777, 12.50000000000000000, -5.737276932171712751 ) ) ;
#110924=EDGE_CURVE ( 'NONE', #44638, #50039, #122635, .T. ) ;
#110925=PLANE ( 'NONE',  #63811 ) ;
#110927=DIRECTION ( 'NONE',  ( 0.000000000000000000, 1.000000000000000000, 0.000000000000000000 ) ) ;
#110928=PLANE ( 'NONE',  #28257 ) ;
#110929=FACE_OUTER_BOUND ( 'NONE', #82842, .T. ) ;
#110930=ORIENTED_EDGE ( 'NONE', *, *, #77254, .T. ) ;
#110931=EDGE_CURVE ( 'NONE', #20474, #13562, #25738, .T. ) ;
#110932=ORIENTED_EDGE ( 'NONE', *, *, #90235, .T. ) ;
#110933=ORIENTED_EDGE ( 'NONE', *, *, #126289, .F. ) ;
#110934=ORIENTED_EDGE ( 'NONE', *, *, #124815, .T. ) ;
#110935=VERTEX_POINT ( 'NONE', #55215 ) ;
#110936=ORIENTED_EDGE ( 'NONE', *, *, #115442, .T. ) ;
#110937=FACE_OUTER_BOUND ( 'NONE', #94017, .T. ) ;
#110938=ORIENTED_EDGE ( 'NONE', *, *, #10809, .T. ) ;
#110939=AXIS2_PLACEMENT_3D ( 'NONE', #22327, #13762, #43899 ) ;
#110940=CIRCLE ( 'NONE', #54511, 0.1000000000000000056 ) ;
#110941=CARTESIAN_POINT ( 'NONE',  ( 11.84999999999990727, 2.500000000000000000, 6.841600689897072485 ) ) ;
#110942=CARTESIAN_POINT ( 'NONE',  ( 14.66596005923785206, -1.500000000000032641, 7.515560522276935274 ) ) ;
#110943=CARTESIAN_POINT ( 'NONE',  ( 12.09999999999990195, 2.500000000000000000, -0.6928203230275541413 ) ) ;
#110944=LINE ( 'NONE', #42237, #84421 ) ;
#110945=ORIENTED_EDGE ( 'NONE', *, *, #21755, .T. ) ;
#110946=PLANE ( 'NONE',  #127930 ) ;
#110947=AXIS2_PLACEMENT_3D ( 'NONE', #8581, #48537, #88441 ) ;
#110948=ORIENTED_EDGE ( 'NONE', *, *, #94914, .T. ) ;
#110949=ORIENTED_EDGE ( 'NONE', *, *, #109076, .F. ) ;
#110950=FACE_OUTER_BOUND ( 'NONE', #59838, .T. ) ;
#110951=CARTESIAN_POINT ( 'NONE',  ( -12.29999999999999538, 2.500000000000000000, -0.3464101615137741841 ) ) ;
#110952=CARTESIAN_POINT ( 'NONE',  ( -9.600000000000008527, 2.500000000000000000, -0.1000000000000023925 ) ) ;
#110954=EDGE_LOOP ( 'NONE', ( #100008, #46485, #14040, #38988 ) ) ;
#110955=ORIENTED_EDGE ( 'NONE', *, *, #46420, .T. ) ;
#110956=AXIS2_PLACEMENT_3D ( 'NONE', #102032, #41837, #63394 ) ;
#110957=EDGE_CURVE ( 'NONE', #3765, #109502, #50864, .T. ) ;
#110958=PLANE ( 'NONE',  #54796 ) ;
#110959=AXIS2_PLACEMENT_3D ( 'NONE', #21387, #101243, #124098 ) ;
#110960=DIRECTION ( 'NONE',  ( 0.000000000000000000, 1.000000000000000000, 0.000000000000000000 ) ) ;
#110961=CARTESIAN_POINT ( 'NONE',  ( -3.100000000000028511, 2.500000000000000000, -3.883716857408426648 ) ) ;
#110962=CARTESIAN_POINT ( 'NONE',  ( 6.649999999999931966, 12.50000000000000000, -7.122917578226816815 ) ) ;
#110963=ORIENTED_EDGE ( 'NONE', *, *, #79658, .F. ) ;
#110964=DIRECTION ( 'NONE',  ( 0.000000000000000000, 1.000000000000000000, 0.000000000000000000 ) ) ;
#110965=AXIS2_PLACEMENT_3D ( 'NONE', #107843, #18167, #87548 ) ;
#110966=ORIENTED_EDGE ( 'NONE', *, *, #39689, .T. ) ;
#110967=CARTESIAN_POINT ( 'NONE',  ( 15.83209681635537258, -2.500000000000000000, 5.404881881984332281 ) ) ;
#110968=ORIENTED_EDGE ( 'NONE', *, *, #101403, .F. ) ;
#110969=CARTESIAN_POINT ( 'NONE',  ( 14.54999999999989591, 12.50000000000000000, 2.165063509461097713 ) ) ;
#110970=CARTESIAN_POINT ( 'NONE',  ( 1.449999999999950440, 2.500000000000000000, 6.048780366869520364 ) ) ;
#110971=AXIS2_PLACEMENT_3D ( 'NONE', #89357, #82774, #111568 ) ;
#110972=DIRECTION ( 'NONE',  ( 0.000000000000000000, 0.000000000000000000, -1.000000000000000000 ) ) ;
#110973=EDGE_CURVE ( 'NONE', #124496, #18418, #71796, .T. ) ;
#110974=EDGE_CURVE ( 'NONE', #104656, #60686, #9760, .T. ) ;
#110975=CARTESIAN_POINT ( 'NONE',  ( -4.600000000000024514, 2.500000000000000000, 0.6928203230275494784 ) ) ;
#110976=EDGE_LOOP ( 'NONE', ( #25674, #111996, #2831, #21730 ) ) ;
#110977=DIRECTION ( 'NONE',  ( 0.000000000000000000, 0.000000000000000000, -1.000000000000000000 ) ) ;
#110978=DIRECTION ( 'NONE',  ( -4.274815082592931898E-19, -0.9999939076577903929, -0.003490651415223739937 ) ) ;
#110979=EDGE_LOOP ( 'NONE', ( #67585, #99569, #81497, #101639 ) ) ;
#110980=EDGE_LOOP ( 'NONE', ( #105834, #121746 ) ) ;
#110981=EDGE_CURVE ( 'NONE', #94678, #28470, #30715, .T. ) ;
#110982=ORIENTED_EDGE ( 'NONE', *, *, #54766, .T. ) ;
#110983=CARTESIAN_POINT ( 'NONE',  ( 17.50000000000000000, -2.750000000000000444, 3.432456362931491700 ) ) ;
#110984=DIRECTION ( 'NONE',  ( 0.000000000000000000, 0.000000000000000000, 1.000000000000000000 ) ) ;
#110985=DIRECTION ( 'NONE',  ( 0.000000000000000000, -0.9999939076577903929, 0.003490651415223739937 ) ) ;
#110986=DIRECTION ( 'NONE',  ( 0.000000000000000000, 1.000000000000000000, 0.000000000000000000 ) ) ;
#110987=DIRECTION ( 'NONE',  ( -0.000000000000000000, 1.000000000000000000, -0.000000000000000000 ) ) ;
#110988=FACE_OUTER_BOUND ( 'NONE', #104179, .T. ) ;
#110989=DIRECTION ( 'NONE',  ( -0.000000000000000000, 1.000000000000000000, -0.000000000000000000 ) ) ;
#110990=CARTESIAN_POINT ( 'NONE',  ( 7.099999999999926814, 2.500000000000000000, -0.7928203230275542301 ) ) ;
#110991=CARTESIAN_POINT ( 'NONE',  ( 6.249999999999930722, 12.50000000000000000, -1.472243186433550122 ) ) ;
#110992=CONICAL_SURFACE ( 'NONE', #96413, 0.09999999999999982514, 0.003490658503988666988 ) ;
#110993=CONICAL_SURFACE ( 'NONE', #23265, 0.1000000000000000472, 0.003490658503988666988 ) ;
#110994=CIRCLE ( 'NONE', #33743, 0.06509327318403741736 ) ;
#110995=AXIS2_PLACEMENT_3D ( 'NONE', #37957, #7191, #37330 ) ;
#110997=FACE_OUTER_BOUND ( 'NONE', #49952, .T. ) ;
#110998=CONICAL_SURFACE ( 'NONE', #21138, 0.09999999999999982514, 0.003490658503988666988 ) ;
#110999=CARTESIAN_POINT ( 'NONE',  ( 13.14999999999989733, 2.500000000000000000, -1.818653347947325916 ) ) ;
#111000=FACE_OUTER_BOUND ( 'NONE', #45320, .T. ) ;
#111001=CARTESIAN_POINT ( 'NONE',  ( -12.29999999999999538, 12.50000000000000000, 4.676537180435972552 ) ) ;
#111003=DIRECTION ( 'NONE',  ( 0.000000000000000000, 0.000000000000000000, -1.000000000000000000 ) ) ;
#111004=ADVANCED_FACE ( 'NONE', ( #101247 ), #101897, .T. ) ;
#111005=FACE_OUTER_BOUND ( 'NONE', #76411, .T. ) ;
#111006=DIRECTION ( 'NONE',  ( 0.000000000000000000, -0.9999939076577903929, 0.003490651415223739937 ) ) ;
#111007=ORIENTED_EDGE ( 'NONE', *, *, #63503, .T. ) ;
#111008=EDGE_CURVE ( 'NONE', #100170, #36170, #110107, .T. ) ;
#111009=EDGE_CURVE ( 'NONE', #81664, #89399, #12209, .T. ) ;
#111010=ORIENTED_EDGE ( 'NONE', *, *, #17607, .F. ) ;
#111011=DIRECTION ( 'NONE',  ( 0.000000000000000000, 1.000000000000000000, 0.000000000000000000 ) ) ;
#111012=ORIENTED_EDGE ( 'NONE', *, *, #93307, .T. ) ;
#111013=ORIENTED_EDGE ( 'NONE', *, *, #58258, .T. ) ;
#111014=PLANE ( 'NONE',  #99151 ) ;
#111015=EDGE_CURVE ( 'NONE', #126895, #121003, #68239, .T. ) ;
#111016=EDGE_CURVE ( 'NONE', #47134, #935, #127187, .T. ) ;
#111017=ADVANCED_FACE ( 'NONE', ( #58443 ), #24429, .T. ) ;
#111018=CARTESIAN_POINT ( 'NONE',  ( -6.050000000000018474, 2.500000000000000000, 6.841600689897072485 ) ) ;
#111019=CARTESIAN_POINT ( 'NONE',  ( 4.799999999999934097, 2.500000000000000000, 4.776537180435972196 ) ) ;
#111020=CARTESIAN_POINT ( 'NONE',  ( 6.449999999999931788, 12.50000000000000000, -2.511473670974877948 ) ) ;
#111021=CIRCLE ( 'NONE', #23211, 0.06509327318403745899 ) ;
#111023=CONICAL_SURFACE ( 'NONE', #127773, 0.1000000000000000472, 0.003490658503988666988 ) ;
#111024=EDGE_CURVE ( 'NONE', #19044, #71330, #107529, .T. ) ;
#111025=DIRECTION ( 'NONE',  ( 0.000000000000000000, 1.000000000000000000, 0.000000000000000000 ) ) ;
#111026=ORIENTED_EDGE ( 'NONE', *, *, #104227, .T. ) ;
#111027=DIRECTION ( 'NONE',  ( -0.000000000000000000, 1.000000000000000000, -0.000000000000000000 ) ) ;
#111028=ADVANCED_FACE ( 'NONE', ( #36223 ), #11810, .T. ) ;
#111029=FACE_OUTER_BOUND ( 'NONE', #52867, .T. ) ;
#111030=ADVANCED_FACE ( 'NONE', ( #78066 ), #17851, .T. ) ;
#111031=ORIENTED_EDGE ( 'NONE', *, *, #70838, .T. ) ;
#111032=CIRCLE ( 'NONE', #14879, 0.06509327318403745899 ) ;
#111033=ORIENTED_EDGE ( 'NONE', *, *, #73767, .T. ) ;
#111034=ORIENTED_EDGE ( 'NONE', *, *, #41304, .F. ) ;
#111035=EDGE_LOOP ( 'NONE', ( #54427, #110303, #41315, #82687 ) ) ;
#111036=PLANE ( 'NONE',  #110959 ) ;
#111037=CARTESIAN_POINT ( 'NONE',  ( 7.180215335589515746, 2.500000000000001332, 8.697219394723591179 ) ) ;
#111038=DIRECTION ( 'NONE',  ( 0.000000000000000000, -0.000000000000000000, 1.000000000000000000 ) ) ;
#111039=FACE_BOUND ( 'NONE', #18631, .T. ) ;
#111040=DIRECTION ( 'NONE',  ( 0.000000000000000000, 1.000000000000000000, 0.000000000000000000 ) ) ;
#111042=PLANE ( 'NONE',  #9233 ) ;
#111043=DIRECTION ( 'NONE',  ( 0.000000000000000000, -0.9999939076577903929, 0.003490651415223739937 ) ) ;
#111044=AXIS2_PLACEMENT_3D ( 'NONE', #3034, #70475, #31214 ) ;
#111045=AXIS2_PLACEMENT_3D ( 'NONE', #40910, #80815, #31082 ) ;
#111046=CIRCLE ( 'NONE', #96478, 0.06509327318403745899 ) ;
#111047=DIRECTION ( 'NONE',  ( 0.000000000000000000, -0.000000000000000000, 1.000000000000000000 ) ) ;
#111048=DIRECTION ( 'NONE',  ( -0.000000000000000000, 1.000000000000000000, -0.000000000000000000 ) ) ;
#111049=DIRECTION ( 'NONE',  ( 0.000000000000000000, -0.9999939076577903929, 0.003490651415223739937 ) ) ;
#111050=VECTOR ( 'NONE', #112997, 1000.000000000000000 ) ;
#111051=CARTESIAN_POINT ( 'NONE',  ( -10.60000000000000320, 2.500000000000000000, -3.883716857408422207 ) ) ;
#111052=ORIENTED_EDGE ( 'NONE', *, *, #9835, .F. ) ;
#111053=AXIS2_PLACEMENT_3D ( 'NONE', #85952, #124615, #104946 ) ;
#111054=AXIS2_PLACEMENT_3D ( 'NONE', #77021, #107771, #18094 ) ;
#111055=ORIENTED_EDGE ( 'NONE', *, *, #56009, .F. ) ;
#111057=ORIENTED_EDGE ( 'NONE', *, *, #102843, .T. ) ;
#111058=VERTEX_POINT ( 'NONE', #76137 ) ;
#111059=FACE_OUTER_BOUND ( 'NONE', #77213, .T. ) ;
#111060=CARTESIAN_POINT ( 'NONE',  ( 2.899999999999945732, 2.500000000000000000, -4.230127018922201998 ) ) ;
#111061=ORIENTED_EDGE ( 'NONE', *, *, #65381, .T. ) ;
#111062=FACE_BOUND ( 'NONE', #120636, .T. ) ;
#111064=EDGE_CURVE ( 'NONE', #34594, #93338, #1345, .T. ) ;
#111065=ADVANCED_FACE ( 'NONE', ( #96402 ), #3503, .T. ) ;
#111066=ORIENTED_EDGE ( 'NONE', *, *, #48262, .T. ) ;
#111067=DIRECTION ( 'NONE',  ( -4.274815082592931898E-19, -0.9999939076577903929, -0.003490651415223739937 ) ) ;
#111068=CARTESIAN_POINT ( 'NONE',  ( 4.999999999999938716, 12.50000000000000000, -5.088040615133791356 ) ) ;
#111069=CARTESIAN_POINT ( 'NONE',  ( 9.399999999999915090, 2.500000000000000000, -4.083716857408426826 ) ) ;
#111070=CARTESIAN_POINT ( 'NONE',  ( -11.84999999999999609, 12.50000000000000000, 6.841600689897072485 ) ) ;
#111071=EDGE_LOOP ( 'NONE', ( #127720, #27001 ) ) ;
#111072=LINE ( 'NONE', #21425, #82665 ) ;
#111073=VERTEX_POINT ( 'NONE', #57134 ) ;
#111074=AXIS2_PLACEMENT_3D ( 'NONE', #83710, #73240, #34624 ) ;
#111075=ORIENTED_EDGE ( 'NONE', *, *, #103771, .T. ) ;
#111076=CIRCLE ( 'NONE', #54653, 0.1000000000000000472 ) ;
#111077=DIRECTION ( 'NONE',  ( 0.000000000000000000, 1.000000000000000000, 0.000000000000000000 ) ) ;
#111078=AXIS2_PLACEMENT_3D ( 'NONE', #117240, #117907, #67501 ) ;
#111080=ORIENTED_EDGE ( 'NONE', *, *, #64808, .T. ) ;
#111081=DIRECTION ( 'NONE',  ( 0.000000000000000000, 0.000000000000000000, 1.000000000000000000 ) ) ;
#111082=DIRECTION ( 'NONE',  ( 0.000000000000000000, 0.000000000000000000, 1.000000000000000000 ) ) ;
#111083=VECTOR ( 'NONE', #83054, 1000.000000000000000 ) ;
#111084=PLANE ( 'NONE',  #49908 ) ;
#111085=CONICAL_SURFACE ( 'NONE', #115189, 0.1000000000000002554, 0.003490658503988666988 ) ;
#111086=CARTESIAN_POINT ( 'NONE',  ( 9.799999999999915445, 2.500000000000000000, 3.983716857408420964 ) ) ;
#111087=PLANE ( 'NONE',  #91481 ) ;
#111088=EDGE_LOOP ( 'NONE', ( #42759, #41569, #48766, #265 ) ) ;
#111089=VECTOR ( 'NONE', #17922, 1000.000000000000000 ) ;
#111090=CARTESIAN_POINT ( 'NONE',  ( 7.499999999999960032, 12.50000000000000000, -0.06509327318403970719 ) ) ;
#111091=ORIENTED_EDGE ( 'NONE', *, *, #2111, .T. ) ;
#111092=DIRECTION ( 'NONE',  ( 0.000000000000000000, 0.000000000000000000, 1.000000000000000000 ) ) ;
#111093=ORIENTED_EDGE ( 'NONE', *, *, #100951, .F. ) ;
#111094=CARTESIAN_POINT ( 'NONE',  ( -6.249999999999981348, 2.500000000000000000, 6.495190528383297135 ) ) ;
#111095=ORIENTED_EDGE ( 'NONE', *, *, #49969, .T. ) ;
#111096=DIRECTION ( 'NONE',  ( 0.000000000000000000, 0.000000000000000000, -1.000000000000000000 ) ) ;
#111097=CARTESIAN_POINT ( 'NONE',  ( -14.99999999999998401, 2.500000000000000000, 0.7928203230275517877 ) ) ;
#111098=FACE_OUTER_BOUND ( 'NONE', #4293, .T. ) ;
#111099=CARTESIAN_POINT ( 'NONE',  ( -14.14999999999998792, 2.500000000000000000, 2.957883832488652942 ) ) ;
#111100=CARTESIAN_POINT ( 'NONE',  ( 17.17279024593002745, 1.352253750625354245, -5.266180533623050053 ) ) ;
#111101=ORIENTED_EDGE ( 'NONE', *, *, #36034, .T. ) ;
#111102=EDGE_LOOP ( 'NONE', ( #23761, #41092 ) ) ;
#111103=EDGE_CURVE ( 'NONE', #86078, #90873, #128477, .T. ) ;
#111104=VERTEX_POINT ( 'NONE', #57792 ) ;
#111106=DIRECTION ( 'NONE',  ( 0.000000000000000000, 0.000000000000000000, -1.000000000000000000 ) ) ;
#111107=PLANE ( 'NONE',  #121194 ) ;
#111108=ORIENTED_EDGE ( 'NONE', *, *, #104320, .T. ) ;
#111109=ORIENTED_EDGE ( 'NONE', *, *, #76254, .F. ) ;
#111110=ORIENTED_EDGE ( 'NONE', *, *, #816, .F. ) ;
#111112=CIRCLE ( 'NONE', #54677, 0.06509327318403745899 ) ;
#111113=EDGE_LOOP ( 'NONE', ( #81358, #67636 ) ) ;
#111114=DIRECTION ( 'NONE',  ( 0.000000000000000000, -0.000000000000000000, 1.000000000000000000 ) ) ;
#111115=EDGE_CURVE ( 'NONE', #86595, #93018, #84968, .T. ) ;
#111116=PLANE ( 'NONE',  #76970 ) ;
#111117=AXIS2_PLACEMENT_3D ( 'NONE', #42106, #2817, #51298 ) ;
#111118=CARTESIAN_POINT ( 'NONE',  ( -1.050000000000038680, 2.500000000000000000, 6.841600689897072485 ) ) ;
#111119=DIRECTION ( 'NONE',  ( -0.000000000000000000, 1.000000000000000000, -0.000000000000000000 ) ) ;
#111120=DIRECTION ( 'NONE',  ( -0.000000000000000000, -1.000000000000000000, -0.000000000000000000 ) ) ;
#111121=CARTESIAN_POINT ( 'NONE',  ( 14.34999999999989662, 12.50000000000000000, 1.818653347947321475 ) ) ;
#111122=DIRECTION ( 'NONE',  ( 0.000000000000000000, -0.000000000000000000, 1.000000000000000000 ) ) ;
#111123=EDGE_CURVE ( 'NONE', #115958, #3256, #34826, .T. ) ;
#111124=EDGE_CURVE ( 'NONE', #37067, #39039, #76660, .T. ) ;
#111125=FACE_OUTER_BOUND ( 'NONE', #94934, .T. ) ;
#111126=AXIS2_PLACEMENT_3D ( 'NONE', #79814, #128944, #108625 ) ;
#111127=EDGE_LOOP ( 'NONE', ( #102544, #111688, #97644, #6623 ) ) ;
#111128=AXIS2_PLACEMENT_3D ( 'NONE', #77825, #98114, #119683 ) ;
#111129=TOROIDAL_SURFACE ( 'NONE', #44538, 9.000000000000001776, 1.000000000000000000 ) ;
#111130=LINE ( 'NONE', #21485, #101055 ) ;
#111131=AXIS2_PLACEMENT_3D ( 'NONE', #6344, #46291, #116315 ) ;
#111132=EDGE_CURVE ( 'NONE', #57912, #40952, #62004, .T. ) ;
#111133=DIRECTION ( 'NONE',  ( 0.000000000000000000, 0.000000000000000000, -1.000000000000000000 ) ) ;
#111134=ORIENTED_EDGE ( 'NONE', *, *, #74976, .F. ) ;
#111135=ORIENTED_EDGE ( 'NONE', *, *, #6706, .F. ) ;
#111136=ADVANCED_FACE ( 'NONE', ( #66306 ), #95444, .T. ) ;
#111138=DIRECTION ( 'NONE',  ( 0.000000000000000000, 1.000000000000000000, 0.000000000000000000 ) ) ;
#111139=DIRECTION ( 'NONE',  ( 0.000000000000000000, 0.000000000000000000, -1.000000000000000000 ) ) ;
#111140=CONICAL_SURFACE ( 'NONE', #98614, 0.1000000000000002554, 0.003490658503988666988 ) ;
#111141=DIRECTION ( 'NONE',  ( 0.000000000000000000, 1.000000000000000000, 0.000000000000000000 ) ) ;
#111142=DIRECTION ( 'NONE',  ( 0.000000000000000000, 0.000000000000000000, 1.000000000000000000 ) ) ;
#111143=CARTESIAN_POINT ( 'NONE',  ( 8.949999999999915801, 12.50000000000000000, -1.883746621131363597 ) ) ;
#111144=FACE_OUTER_BOUND ( 'NONE', #114660, .T. ) ;
#111145=VECTOR ( 'NONE', #95056, 1000.000000000000000 ) ;
#111146=CARTESIAN_POINT ( 'NONE',  ( -1.700000000000034817, 12.50000000000000000, -4.330127018922201643 ) ) ;
#111147=AXIS2_PLACEMENT_3D ( 'NONE', #65866, #3096, #14803 ) ;
#111148=VECTOR ( 'NONE', #37020, 1000.000000000000000 ) ;
#111149=DIRECTION ( 'NONE',  ( 0.000000000000000000, -0.000000000000000000, 1.000000000000000000 ) ) ;
#111150=ORIENTED_EDGE ( 'NONE', *, *, #62068, .F. ) ;
#111151=ORIENTED_EDGE ( 'NONE', *, *, #117794, .F. ) ;
#111152=CONICAL_SURFACE ( 'NONE', #21285, 0.1000000000000000472, 0.003490658503988666988 ) ;
#111153=ORIENTED_EDGE ( 'NONE', *, *, #76617, .T. ) ;
#111154=ORIENTED_EDGE ( 'NONE', *, *, #102812, .F. ) ;
#111155=DIRECTION ( 'NONE',  ( 0.000000000000000000, -0.9999939076577903929, 0.003490651415223739937 ) ) ;
#111156=FACE_OUTER_BOUND ( 'NONE', #63051, .T. ) ;
#111157=ORIENTED_EDGE ( 'NONE', *, *, #91573, .T. ) ;
#111159=EDGE_CURVE ( 'NONE', #110110, #127840, #13953, .T. ) ;
#111160=DIRECTION ( 'NONE',  ( -0.000000000000000000, 1.000000000000000000, -0.000000000000000000 ) ) ;
#111161=FACE_OUTER_BOUND ( 'NONE', #23381, .T. ) ;
#111162=CARTESIAN_POINT ( 'NONE',  ( 7.699999999999923794, 2.500000000000000000, -0.3464101615137783474 ) ) ;
#111163=VERTEX_POINT ( 'NONE', #56478 ) ;
#111164=EDGE_CURVE ( 'NONE', #119116, #66538, #72463, .T. ) ;
#111165=DIRECTION ( 'NONE',  ( -0.000000000000000000, -1.000000000000000000, -0.000000000000000000 ) ) ;
#111166=ADVANCED_FACE ( 'NONE', ( #15908 ), #6083, .T. ) ;
#111167=DIRECTION ( 'NONE',  ( 0.000000000000000000, 0.000000000000000000, 1.000000000000000000 ) ) ;
#111168=ORIENTED_EDGE ( 'NONE', *, *, #1340, .F. ) ;
#111169=EDGE_LOOP ( 'NONE', ( #117333, #59069, #34429, #105287 ) ) ;
#111170=VERTEX_POINT ( 'NONE', #17180 ) ;
#111173=CARTESIAN_POINT ( 'NONE',  ( 6.649999999999930189, 2.500000000000000000, 5.802370205355744659 ) ) ;
#111175=ADVANCED_FACE ( 'NONE', ( #47327 ), #76755, .T. ) ;
#111176=AXIS2_PLACEMENT_3D ( 'NONE', #32138, #39390, #21000 ) ;
#111177=EDGE_CURVE ( 'NONE', #23570, #44909, #82748, .T. ) ;
#111178=EDGE_CURVE ( 'NONE', #94583, #45538, #106000, .T. ) ;
#111179=EDGE_CURVE ( 'NONE', #102327, #65030, #72562, .T. ) ;
#111180=CARTESIAN_POINT ( 'NONE',  ( -8.100000000000010303, 2.500000000000000000, 4.676537180435972552 ) ) ;
#111181=DIRECTION ( 'NONE',  ( 0.000000000000000000, 0.000000000000000000, 1.000000000000000000 ) ) ;
#111182=AXIS2_PLACEMENT_3D ( 'NONE', #23153, #122649, #102996 ) ;
#111183=VERTEX_POINT ( 'NONE', #61663 ) ;
#111184=CIRCLE ( 'NONE', #113338, 0.1000000000000002554 ) ;
#111185=CIRCLE ( 'NONE', #38052, 0.09999999999999982514 ) ;
#111186=EDGE_CURVE ( 'NONE', #51434, #120113, #49576, .T. ) ;
#111187=LINE ( 'NONE', #30738, #20990 ) ;
#111188=VERTEX_POINT ( 'NONE', #101578 ) ;
#111189=LINE ( 'NONE', #28791, #116396 ) ;
#111190=DIRECTION ( 'NONE',  ( -4.274815082592931898E-19, -0.9999939076577903929, -0.003490651415223739937 ) ) ;
#111191=CIRCLE ( 'NONE', #50557, 0.1000000000000002554 ) ;
#111192=CARTESIAN_POINT ( 'NONE',  ( 10.84999999999991260, 2.500000000000000000, 7.288010851410849256 ) ) ;
#111193=PLANE ( 'NONE',  #40054 ) ;
#111194=EDGE_CURVE ( 'NONE', #68417, #115797, #68341, .T. ) ;
#111195=VECTOR ( 'NONE', #87410, 1000.000000000000000 ) ;
#111196=ORIENTED_EDGE ( 'NONE', *, *, #82750, .T. ) ;
#111197=EDGE_CURVE ( 'NONE', #112193, #47787, #49272, .T. ) ;
#111198=ORIENTED_EDGE ( 'NONE', *, *, #18761, .T. ) ;
#111199=ORIENTED_EDGE ( 'NONE', *, *, #35223, .T. ) ;
#111200=DIRECTION ( 'NONE',  ( -0.000000000000000000, -1.000000000000000000, -0.000000000000000000 ) ) ;
#111201=DIRECTION ( 'NONE',  ( 0.000000000000000000, 1.000000000000000000, 0.000000000000000000 ) ) ;
#111202=FACE_BOUND ( 'NONE', #117749, .T. ) ;
#111203=DIRECTION ( 'NONE',  ( 0.000000000000000000, -0.000000000000000000, 1.000000000000000000 ) ) ;
#111204=DIRECTION ( 'NONE',  ( 0.000000000000000000, -0.9999939076577903929, 0.003490651415223739937 ) ) ;
#111205=PLANE ( 'NONE',  #129465 ) ;
#111206=CARTESIAN_POINT ( 'NONE',  ( 0.5999999999999621192, 12.50000000000000000, 0.3464101615137758494 ) ) ;
#111207=FACE_OUTER_BOUND ( 'NONE', #125047, .T. ) ;
#111209=ORIENTED_EDGE ( 'NONE', *, *, #100783, .F. ) ;
#111210=CONICAL_SURFACE ( 'NONE', #125790, 0.1000000000000002554, 0.003490658503988666988 ) ;
#111211=CARTESIAN_POINT ( 'NONE',  ( 8.949999999999917577, 12.50000000000000000, -2.511473670974877948 ) ) ;
#111212=DIRECTION ( 'NONE',  ( 0.000000000000000000, 1.000000000000000000, 0.000000000000000000 ) ) ;
#111213=ORIENTED_EDGE ( 'NONE', *, *, #73201, .F. ) ;
#111214=ORIENTED_EDGE ( 'NONE', *, *, #51381, .F. ) ;
#111215=CARTESIAN_POINT ( 'NONE',  ( 9.599999999999914380, 2.500000000000000000, 4.330127018922196314 ) ) ;
#111216=CARTESIAN_POINT ( 'NONE',  ( 5.849999999999934808, 12.50000000000000000, -5.802370205355749988 ) ) ;
#111217=FACE_BOUND ( 'NONE', #126349, .T. ) ;
#111218=AXIS2_PLACEMENT_3D ( 'NONE', #106539, #75786, #56772 ) ;
#111219=DIRECTION ( 'NONE',  ( -0.000000000000000000, -1.000000000000000000, -0.000000000000000000 ) ) ;
#111220=AXIS2_PLACEMENT_3D ( 'NONE', #77372, #117256, #67519 ) ;
#111221=AXIS2_PLACEMENT_3D ( 'NONE', #35058, #82863, #22654 ) ;
#111222=ADVANCED_FACE ( 'NONE', ( #133 ), #16086, .T. ) ;
#111223=ORIENTED_EDGE ( 'NONE', *, *, #104214, .F. ) ;
#111224=CARTESIAN_POINT ( 'NONE',  ( -10.00000000000000711, 2.500000000000000000, -3.537306695894645969 ) ) ;
#111226=ORIENTED_EDGE ( 'NONE', *, *, #60280, .F. ) ;
#111227=AXIS2_PLACEMENT_3D ( 'NONE', #104750, #6530, #47801 ) ;
#111228=CARTESIAN_POINT ( 'NONE',  ( 11.89999999999990443, 2.500000000000000000, 0.4464101615137736623 ) ) ;
#111229=DIRECTION ( 'NONE',  ( 0.000000000000000000, -0.000000000000000000, 1.000000000000000000 ) ) ;
#111230=VECTOR ( 'NONE', #45243, 1000.000000000000000 ) ;
#111231=ADVANCED_FACE ( 'NONE', ( #119273 ), #108042, .T. ) ;
#111232=VECTOR ( 'NONE', #113898, 1000.000000000000000 ) ;
#111233=CONICAL_SURFACE ( 'NONE', #50617, 0.1000000000000002554, 0.003490658503988666988 ) ;
#111234=CARTESIAN_POINT ( 'NONE',  ( 0.7999999999999612976, 12.50000000000000000, -1.084202172485504434E-16 ) ) ;
#111236=AXIS2_PLACEMENT_3D ( 'NONE', #30125, #54709, #60854 ) ;
#111237=EDGE_LOOP ( 'NONE', ( #8982, #94172, #77515, #100829 ) ) ;
#111238=CARTESIAN_POINT ( 'NONE',  ( 2.499999999999948930, 12.50000000000000000, -0.6928203230275541413 ) ) ;
#111239=DIRECTION ( 'NONE',  ( 0.000000000000000000, 0.000000000000000000, -1.000000000000000000 ) ) ;
#111240=FACE_OUTER_BOUND ( 'NONE', #75137, .T. ) ;
#111241=ORIENTED_EDGE ( 'NONE', *, *, #98643, .F. ) ;
#111242=ORIENTED_EDGE ( 'NONE', *, *, #108108, .F. ) ;
#111243=PLANE ( 'NONE',  #55540 ) ;
#111244=ORIENTED_EDGE ( 'NONE', *, *, #17652, .F. ) ;
#111245=DIRECTION ( 'NONE',  ( -0.000000000000000000, -1.000000000000000000, -0.000000000000000000 ) ) ;
#111246=DIRECTION ( 'NONE',  ( 0.000000000000000000, 1.000000000000000000, 0.000000000000000000 ) ) ;
#111247=LINE ( 'NONE', #14816, #21643 ) ;
#111248=ORIENTED_EDGE ( 'NONE', *, *, #80313, .T. ) ;
#111249=CARTESIAN_POINT ( 'NONE',  ( 5.399999999999931966, 12.50000000000000000, 4.395220292106234439 ) ) ;
#111250=DIRECTION ( 'NONE',  ( 0.000000000000000000, -0.9999939076577903929, 0.003490651415223739937 ) ) ;
#111251=DIRECTION ( 'NONE',  ( -0.000000000000000000, -1.000000000000000000, -0.000000000000000000 ) ) ;
#111252=FACE_OUTER_BOUND ( 'NONE', #66067, .T. ) ;
#111253=LINE ( 'NONE', #82482, #61179 ) ;
#111254=DIRECTION ( 'NONE',  ( 0.000000000000000000, 1.000000000000000000, 0.000000000000000000 ) ) ;
#111255=ORIENTED_EDGE ( 'NONE', *, *, #91670, .T. ) ;
#111256=VERTEX_POINT ( 'NONE', #10591 ) ;
#111257=CARTESIAN_POINT ( 'NONE',  ( 0.5999999999999621192, 2.500000000000000000, 0.4464101615137758272 ) ) ;
#111258=ORIENTED_EDGE ( 'NONE', *, *, #123193, .F. ) ;
#111259=VECTOR ( 'NONE', #29945, 1000.000000000000000 ) ;
#111260=DIRECTION ( 'NONE',  ( 0.000000000000000000, 1.000000000000000000, 0.000000000000000000 ) ) ;
#111261=AXIS2_PLACEMENT_3D ( 'NONE', #8007, #127161, #7357 ) ;
#111262=CIRCLE ( 'NONE', #98661, 0.06509327318403745899 ) ;
#111263=ORIENTED_EDGE ( 'NONE', *, *, #66266, .T. ) ;
#111264=VERTEX_POINT ( 'NONE', #70187 ) ;
#111265=VERTEX_POINT ( 'NONE', #19797 ) ;
#111266=CARTESIAN_POINT ( 'NONE',  ( 2.699999999999945555, 12.50000000000000000, 4.048810130592458201 ) ) ;
#111267=CARTESIAN_POINT ( 'NONE',  ( 1.249999999999952038, 2.500000000000000000, 5.902370205355745192 ) ) ;
#111268=ADVANCED_FACE ( 'NONE', ( #59745 ), #15817, .T. ) ;
#111269=AXIS2_PLACEMENT_3D ( 'NONE', #125631, #83160, #85712 ) ;
#111270=AXIS2_PLACEMENT_3D ( 'NONE', #83030, #103306, #22824 ) ;
#111271=DIRECTION ( 'NONE',  ( 0.000000000000000000, 1.000000000000000000, 0.000000000000000000 ) ) ;
#111272=AXIS2_PLACEMENT_3D ( 'NONE', #1975, #63491, #111953 ) ;
#111274=CARTESIAN_POINT ( 'NONE',  ( -1.250000000000001110, 2.500000000000000000, -2.165063509461101710 ) ) ;
#111275=DIRECTION ( 'NONE',  ( 0.000000000000000000, -0.9999939076577903929, 0.003490651415223739937 ) ) ;
#111276=CARTESIAN_POINT ( 'NONE',  ( 13.09999999999989839, 2.500000000000000000, -0.2464101615137783419 ) ) ;
#111277=AXIS2_PLACEMENT_3D ( 'NONE', #60439, #61050, #111430 ) ;
#111278=DIRECTION ( 'NONE',  ( 0.000000000000000000, 1.000000000000000000, 0.000000000000000000 ) ) ;
#111279=FACE_OUTER_BOUND ( 'NONE', #61004, .T. ) ;
#111280=ADVANCED_FACE ( 'NONE', ( #80657 ), #9849, .T. ) ;
#111281=EDGE_CURVE ( 'NONE', #46427, #9874, #11247, .T. ) ;
#111282=DIRECTION ( 'NONE',  ( -4.274815082592931898E-19, -0.9999939076577903929, -0.003490651415223739937 ) ) ;
#111283=AXIS2_PLACEMENT_3D ( 'NONE', #41807, #33893, #83012 ) ;
#111284=ORIENTED_EDGE ( 'NONE', *, *, #91078, .F. ) ;
#111286=CARTESIAN_POINT ( 'NONE',  ( 4.349999999999939249, 2.500000000000000000, 2.411473670974873862 ) ) ;
#111287=EDGE_LOOP ( 'NONE', ( #14589, #17477, #104831, #28085 ) ) ;
#111288=ORIENTED_EDGE ( 'NONE', *, *, #87493, .T. ) ;
#111289=EDGE_CURVE ( 'NONE', #73490, #93190, #88990, .T. ) ;
#111290=DIRECTION ( 'NONE',  ( 0.000000000000000000, 1.000000000000000000, 0.000000000000000000 ) ) ;
#111291=CARTESIAN_POINT ( 'NONE',  ( -10.20000000000000462, 12.50000000000000000, -4.741630453620010677 ) ) ;
#111292=AXIS2_PLACEMENT_3D ( 'NONE', #111018, #71116, #110391 ) ;
#111293=DIRECTION ( 'NONE',  ( -0.000000000000000000, -1.000000000000000000, -0.000000000000000000 ) ) ;
#111294=DIRECTION ( 'NONE',  ( 0.000000000000000000, 0.000000000000000000, 1.000000000000000000 ) ) ;
#111295=CARTESIAN_POINT ( 'NONE',  ( -2.300000000000032685, 12.50000000000000000, -4.676537180435978769 ) ) ;
#111296=CARTESIAN_POINT ( 'NONE',  ( 6.899999999999928413, 2.500000000000000000, -4.576537180435977348 ) ) ;
#111297=ORIENTED_EDGE ( 'NONE', *, *, #32744, .T. ) ;
#111298=CONICAL_SURFACE ( 'NONE', #54878, 0.1000000000000002554, 0.003490658503988666988 ) ;
#111299=VERTEX_POINT ( 'NONE', #49918 ) ;
#111300=CIRCLE ( 'NONE', #8906, 0.06509327318403745899 ) ;
#111301=ORIENTED_EDGE ( 'NONE', *, *, #11035, .F. ) ;
#111302=CARTESIAN_POINT ( 'NONE',  ( 5.849999999999932143, 2.500000000000000000, 1.472243186433545459 ) ) ;
#111303=ORIENTED_EDGE ( 'NONE', *, *, #70974, .F. ) ;
#111304=VERTEX_POINT ( 'NONE', #50529 ) ;
#111306=CARTESIAN_POINT ( 'NONE',  ( 13.94999999999989271, 2.500000000000000000, -1.718653347947326049 ) ) ;
#111307=DIRECTION ( 'NONE',  ( 0.000000000000000000, 0.000000000000000000, 1.000000000000000000 ) ) ;
#111308=AXIS2_PLACEMENT_3D ( 'NONE', #127257, #106314, #98409 ) ;
#111309=CIRCLE ( 'NONE', #77870, 0.1000000000000000056 ) ;
#111310=DIRECTION ( 'NONE',  ( 0.000000000000000000, 0.000000000000000000, 1.000000000000000000 ) ) ;
#111311=VECTOR ( 'NONE', #10088, 1000.000000000000000 ) ;
#111313=DIRECTION ( 'NONE',  ( 0.000000000000000000, 1.000000000000000000, 0.000000000000000000 ) ) ;
#111314=EDGE_LOOP ( 'NONE', ( #128072, #122407, #68827, #56968 ) ) ;
#111315=DIRECTION ( 'NONE',  ( -0.000000000000000000, -1.000000000000000000, -0.000000000000000000 ) ) ;
#111316=DIRECTION ( 'NONE',  ( -4.274815082592931898E-19, -0.9999939076577903929, -0.003490651415223739937 ) ) ;
#111317=DIRECTION ( 'NONE',  ( 0.000000000000000000, 0.000000000000000000, 1.000000000000000000 ) ) ;
#111318=DIRECTION ( 'NONE',  ( 0.000000000000000000, 1.000000000000000000, 0.000000000000000000 ) ) ;
#111319=AXIS2_PLACEMENT_3D ( 'NONE', #94158, #62782, #22867 ) ;
#111320=ORIENTED_EDGE ( 'NONE', *, *, #50731, .T. ) ;
#111322=CIRCLE ( 'NONE', #54904, 0.06509327318403745899 ) ;
#111323=VERTEX_POINT ( 'NONE', #121854 ) ;
#111324=EDGE_LOOP ( 'NONE', ( #121371, #18010, #83464, #6507 ) ) ;
#111325=EDGE_CURVE ( 'NONE', #51506, #16102, #70819, .T. ) ;
#111326=CARTESIAN_POINT ( 'NONE',  ( 5.199999999999935341, 12.50000000000000000, -0.3464101615137783474 ) ) ;
#111327=EDGE_CURVE ( 'NONE', #83416, #48128, #81295, .T. ) ;
#111328=CONICAL_SURFACE ( 'NONE', #4720, 0.1000000000000002554, 0.003490658503988666988 ) ;
#111329=ADVANCED_FACE ( 'NONE', ( #32214 ), #66285, .T. ) ;
#111330=ORIENTED_EDGE ( 'NONE', *, *, #95147, .F. ) ;
#111331=DIRECTION ( 'NONE',  ( 0.000000000000000000, 0.000000000000000000, 1.000000000000000000 ) ) ;
#111332=DIRECTION ( 'NONE',  ( 0.000000000000000000, 0.000000000000000000, 1.000000000000000000 ) ) ;
#111333=VECTOR ( 'NONE', #47684, 1000.000000000000000 ) ;
#111334=EDGE_CURVE ( 'NONE', #1500, #18199, #26306, .T. ) ;
#111335=ORIENTED_EDGE ( 'NONE', *, *, #72479, .T. ) ;
#111336=CARTESIAN_POINT ( 'NONE',  ( 0.5999999999999560130, 2.500000000000000000, -4.083716857408426826 ) ) ;
#111337=DIRECTION ( 'NONE',  ( -0.000000000000000000, -1.000000000000000000, -0.000000000000000000 ) ) ;
#111338=CARTESIAN_POINT ( 'NONE',  ( -1.050000000000037348, 12.50000000000000000, -2.511473670974877948 ) ) ;
#111339=CARTESIAN_POINT ( 'NONE',  ( 8.949999999999917577, 12.50000000000000000, 6.148780366869520009 ) ) ;
#111340=EDGE_CURVE ( 'NONE', #55154, #99389, #26583, .T. ) ;
#111341=EDGE_CURVE ( 'NONE', #122246, #22448, #34135, .T. ) ;
#111342=CARTESIAN_POINT ( 'NONE',  ( 7.499999999999923617, 2.500000000000000000, 0.6928203230275494784 ) ) ;
#111343=ORIENTED_EDGE ( 'NONE', *, *, #102912, .T. ) ;
#111344=CONICAL_SURFACE ( 'NONE', #65390, 0.1000000000000000472, 0.003490658503988666988 ) ;
#111345=ORIENTED_EDGE ( 'NONE', *, *, #83451, .T. ) ;
#111346=AXIS2_PLACEMENT_3D ( 'NONE', #65449, #43266, #24892 ) ;
#111347=CARTESIAN_POINT ( 'NONE',  ( 7.299999999999924327, 12.50000000000000000, 0.2813168883297361700 ) ) ;
#111348=CARTESIAN_POINT ( 'NONE',  ( 1.649999999999951950, 12.50000000000000000, -5.802370205355749988 ) ) ;
#111349=EDGE_CURVE ( 'NONE', #4289, #32314, #104773, .T. ) ;
#111350=CARTESIAN_POINT ( 'NONE',  ( 6.849999999999927702, 2.500000000000000000, 2.611473670974873151 ) ) ;
#111351=DIRECTION ( 'NONE',  ( 0.000000000000000000, -0.9999939076577903929, 0.003490651415223739937 ) ) ;
#111352=ORIENTED_EDGE ( 'NONE', *, *, #17830, .T. ) ;
#111353=CIRCLE ( 'NONE', #94639, 0.06509327318403745899 ) ;
#111354=CIRCLE ( 'NONE', #48598, 0.06509327318403741736 ) ;
#111355=CIRCLE ( 'NONE', #38238, 0.06509327318403745899 ) ;
#111356=ORIENTED_EDGE ( 'NONE', *, *, #129164, .F. ) ;
#111357=DIRECTION ( 'NONE',  ( -0.000000000000000000, -1.000000000000000000, -0.000000000000000000 ) ) ;
#111358=PLANE ( 'NONE',  #30041 ) ;
#111359=CARTESIAN_POINT ( 'NONE',  ( 8.749999999999920064, 2.500000000000000000, 5.902370205355745192 ) ) ;
#111360=PLANE ( 'NONE',  #11238 ) ;
#111361=VERTEX_POINT ( 'NONE', #82592 ) ;
#111362=CIRCLE ( 'NONE', #23649, 0.1000000000000002554 ) ;
#111363=DIRECTION ( 'NONE',  ( 0.000000000000000000, 0.000000000000000000, -1.000000000000000000 ) ) ;
#111364=CIRCLE ( 'NONE', #25704, 0.06509327318403745899 ) ;
#111365=CONICAL_SURFACE ( 'NONE', #128118, 0.1000000000000002554, 0.003490658503988666988 ) ;
#111366=CARTESIAN_POINT ( 'NONE',  ( 8.749999999999923617, 12.50000000000000000, -7.188010851410854052 ) ) ;
#111367=AXIS2_PLACEMENT_3D ( 'NONE', #112746, #23071, #13227 ) ;
#111368=VERTEX_POINT ( 'NONE', #93053 ) ;
#111369=CIRCLE ( 'NONE', #75886, 0.1000000000000002554 ) ;
#111370=DIRECTION ( 'NONE',  ( 0.000000000000000000, 0.000000000000000000, -1.000000000000000000 ) ) ;
#111371=ADVANCED_FACE ( 'NONE', ( #64860 ), #124441, .T. ) ;
#111372=VERTEX_POINT ( 'NONE', #12536 ) ;
#111373=AXIS2_PLACEMENT_3D ( 'NONE', #20704, #13442, #50810 ) ;
#111374=DIRECTION ( 'NONE',  ( 0.000000000000000000, 0.000000000000000000, -1.000000000000000000 ) ) ;
#111375=VERTEX_POINT ( 'NONE', #94316 ) ;
#111376=ORIENTED_EDGE ( 'NONE', *, *, #116372, .T. ) ;
#111377=DIRECTION ( 'NONE',  ( 0.000000000000000000, 0.000000000000000000, 1.000000000000000000 ) ) ;
#111378=DIRECTION ( 'NONE',  ( 0.000000000000000000, 1.000000000000000000, 0.000000000000000000 ) ) ;
#111379=EDGE_LOOP ( 'NONE', ( #121244, #121804 ) ) ;
#111380=ORIENTED_EDGE ( 'NONE', *, *, #13493, .F. ) ;
#111381=DIRECTION ( 'NONE',  ( 0.000000000000000000, -0.000000000000000000, 1.000000000000000000 ) ) ;
#111382=DIRECTION ( 'NONE',  ( 0.000000000000000000, 1.000000000000000000, 0.000000000000000000 ) ) ;
#111383=ORIENTED_EDGE ( 'NONE', *, *, #115236, .F. ) ;
#111384=CIRCLE ( 'NONE', #61241, 0.06509327318403745899 ) ;
#111385=DIRECTION ( 'NONE',  ( 0.000000000000000000, 0.000000000000000000, 1.000000000000000000 ) ) ;
#111387=ADVANCED_FACE ( 'NONE', ( #85150 ), #62309, .T. ) ;
#111388=CARTESIAN_POINT ( 'NONE',  ( -14.99999999999998224, 12.50000000000000000, -0.6928203230275519209 ) ) ;
#111389=CARTESIAN_POINT ( 'NONE',  ( 6.049999999999930544, 2.500000000000000000, 2.411473670974873862 ) ) ;
#111390=CARTESIAN_POINT ( 'NONE',  ( -14.14999999999998614, 2.500000000000000000, 2.265063509461101354 ) ) ;
#111391=CARTESIAN_POINT ( 'NONE',  ( -1.850000000000033840, 2.500000000000000000, 6.941600689897073018 ) ) ;
#111392=DIRECTION ( 'NONE',  ( 0.000000000000000000, -0.9999939076577903929, 0.003490651415223739937 ) ) ;
#111393=AXIS2_PLACEMENT_3D ( 'NONE', #45370, #5418, #49725 ) ;
#111394=CIRCLE ( 'NONE', #19367, 0.06509327318403745899 ) ;
#111395=CIRCLE ( 'NONE', #38271, 0.06509327318403745899 ) ;
#111396=ORIENTED_EDGE ( 'NONE', *, *, #121855, .T. ) ;
#111397=ORIENTED_EDGE ( 'NONE', *, *, #24558, .T. ) ;
#111398=CARTESIAN_POINT ( 'NONE',  ( 13.74999999999993072, 12.50000000000000000, -2.165063509461101710 ) ) ;
#111399=ORIENTED_EDGE ( 'NONE', *, *, #33064, .F. ) ;
#111400=DIRECTION ( 'NONE',  ( 0.000000000000000000, 1.000000000000000000, 0.000000000000000000 ) ) ;
#111401=DIRECTION ( 'NONE',  ( -0.000000000000000000, 1.000000000000000000, -0.000000000000000000 ) ) ;
#111402=DIRECTION ( 'NONE',  ( -0.000000000000000000, 1.000000000000000000, -0.000000000000000000 ) ) ;
#111403=ORIENTED_EDGE ( 'NONE', *, *, #122447, .F. ) ;
#111404=ORIENTED_EDGE ( 'NONE', *, *, #115747, .F. ) ;
#111405=FACE_BOUND ( 'NONE', #39259, .T. ) ;
#111406=ORIENTED_EDGE ( 'NONE', *, *, #11097, .F. ) ;
#111407=DIRECTION ( 'NONE',  ( 0.000000000000000000, 0.000000000000000000, 1.000000000000000000 ) ) ;
#111408=CARTESIAN_POINT ( 'NONE',  ( 7.499999999999960032, 12.50000000000000000, -2.276824562219559311E-15 ) ) ;
#111409=AXIS2_PLACEMENT_3D ( 'NONE', #74775, #43395, #102933 ) ;
#111410=CIRCLE ( 'NONE', #121892, 0.1000000000000002554 ) ;
#111411=LINE ( 'NONE', #21771, #128497 ) ;
#111412=DIRECTION ( 'NONE',  ( -0.000000000000000000, -1.000000000000000000, -0.000000000000000000 ) ) ;
#111413=CIRCLE ( 'NONE', #92651, 0.06509327318403745899 ) ;
#111414=LINE ( 'NONE', #21773, #120411 ) ;
#111415=CARTESIAN_POINT ( 'NONE',  ( 12.89999999999989733, 2.500000000000000000, -2.385244779468109755E-15 ) ) ;
#111416=DIRECTION ( 'NONE',  ( -0.000000000000000000, -1.000000000000000000, -0.000000000000000000 ) ) ;
#111417=CARTESIAN_POINT ( 'NONE',  ( 2.899999999999945732, 2.500000000000000000, -0.1000000000000023925 ) ) ;
#111418=LINE ( 'NONE', #101630, #105975 ) ;
#111419=LINE ( 'NONE', #112089, #92478 ) ;
#111420=CIRCLE ( 'NONE', #54996, 0.1000000000000002554 ) ;
#111421=CARTESIAN_POINT ( 'NONE',  ( -2.900000000000030109, 2.500000000000000000, 0.6928203230275494784 ) ) ;
#111422=ORIENTED_EDGE ( 'NONE', *, *, #102356, .F. ) ;
#111423=ORIENTED_EDGE ( 'NONE', *, *, #99973, .F. ) ;
#111424=VERTEX_POINT ( 'NONE', #32857 ) ;
#111425=AXIS2_PLACEMENT_3D ( 'NONE', #92813, #71218, #3137 ) ;
#111426=ORIENTED_EDGE ( 'NONE', *, *, #119909, .F. ) ;
#111427=CIRCLE ( 'NONE', #100976, 0.06509327318403745899 ) ;
#111428=CIRCLE ( 'NONE', #126104, 0.06509327318403745899 ) ;
#111429=CARTESIAN_POINT ( 'NONE',  ( -6.850000000000013856, 2.500000000000000000, 6.048780366869521252 ) ) ;
#111430=DIRECTION ( 'NONE',  ( 0.000000000000000000, -0.000000000000000000, 1.000000000000000000 ) ) ;
#111431=ORIENTED_EDGE ( 'NONE', *, *, #98624, .T. ) ;
#111432=EDGE_LOOP ( 'NONE', ( #25544, #121283, #117762, #116183 ) ) ;
#111433=EDGE_LOOP ( 'NONE', ( #73143, #22921 ) ) ;
#111434=VECTOR ( 'NONE', #36412, 1000.000000000000000 ) ;
#111435=CARTESIAN_POINT ( 'NONE',  ( -9.550000000000002487, 12.50000000000000000, 6.495190528383297135 ) ) ;
#111436=EDGE_CURVE ( 'NONE', #60385, #4249, #4633, .T. ) ;
#111437=DIRECTION ( 'NONE',  ( -0.000000000000000000, 1.000000000000000000, -0.000000000000000000 ) ) ;
#111438=CIRCLE ( 'NONE', #55006, 0.1000000000000000056 ) ;
#111439=SURFACE_SIDE_STYLE ('',( #81367 ) ) ;
#111440=FACE_OUTER_BOUND ( 'NONE', #70771, .T. ) ;
#111441=LINE ( 'NONE', #91818, #68024 ) ;
#111442=CARTESIAN_POINT ( 'NONE',  ( -10.85000000000000142, 12.50000000000000000, 2.165063509461097713 ) ) ;
#111443=CARTESIAN_POINT ( 'NONE',  ( 3.749999999999938716, 2.500000000000000000, 7.188010851410848723 ) ) ;
#111444=ADVANCED_FACE ( 'NONE', ( #114605 ), #60049, .T. ) ;
#111445=ORIENTED_EDGE ( 'NONE', *, *, #101596, .F. ) ;
#111446=EDGE_CURVE ( 'NONE', #25426, #106311, #1429, .T. ) ;
#111447=CARTESIAN_POINT ( 'NONE',  ( 8.349999999999923261, 2.500000000000000000, 2.757883832488649656 ) ) ;
#111448=VERTEX_POINT ( 'NONE', #112046 ) ;
#111449=ORIENTED_EDGE ( 'NONE', *, *, #123420, .T. ) ;
#111450=ORIENTED_EDGE ( 'NONE', *, *, #109888, .F. ) ;
#111451=EDGE_CURVE ( 'NONE', #49607, #66867, #32580, .T. ) ;
#111452=CARTESIAN_POINT ( 'NONE',  ( -6.250000000000021316, 2.500000000000000000, -5.802370205355749988 ) ) ;
#111453=EDGE_CURVE ( 'NONE', #82216, #56145, #112269, .T. ) ;
#111454=CIRCLE ( 'NONE', #9048, 0.1000000000000002554 ) ;
#111455=ADVANCED_FACE ( 'NONE', ( #52465 ), #78832, .T. ) ;
#111456=ORIENTED_EDGE ( 'NONE', *, *, #38060, .F. ) ;
#111457=EDGE_LOOP ( 'NONE', ( #117315, #64072, #7826, #28091 ) ) ;
#111458=EDGE_CURVE ( 'NONE', #40679, #93080, #5628, .T. ) ;
#111459=ADVANCED_FACE ( 'NONE', ( #112692 ), #53127, .T. ) ;
#111460=ORIENTED_EDGE ( 'NONE', *, *, #39420, .F. ) ;
#111461=CARTESIAN_POINT ( 'NONE',  ( 6.649999999999929301, 12.50000000000000000, 6.495190528383297135 ) ) ;
#111462=VECTOR ( 'NONE', #128627, 1000.000000000000000 ) ;
#111463=FACE_OUTER_BOUND ( 'NONE', #58956, .T. ) ;
#111464=PLANE ( 'NONE',  #93920 ) ;
#111465=CONICAL_SURFACE ( 'NONE', #55029, 0.1000000000000002554, 0.003490658503988666988 ) ;
#111466=DIRECTION ( 'NONE',  ( -0.000000000000000000, 1.000000000000000000, -0.000000000000000000 ) ) ;
#111467=DIRECTION ( 'NONE',  ( 0.000000000000000000, 1.000000000000000000, 0.000000000000000000 ) ) ;
#111468=AXIS2_PLACEMENT_3D ( 'NONE', #39829, #119645, #69917 ) ;
#111469=AXIS2_PLACEMENT_3D ( 'NONE', #73013, #11511, #51456 ) ;
#111470=LINE ( 'NONE', #31014, #106838 ) ;
#111471=ADVANCED_FACE ( 'NONE', ( #33498 ), #93484, .T. ) ;
#111472=CARTESIAN_POINT ( 'NONE',  ( -3.350000000000028511, 2.500000000000000000, -1.472243186433550122 ) ) ;
#111473=AXIS2_PLACEMENT_3D ( 'NONE', #11209, #51159, #112648 ) ;
#111474=CONICAL_SURFACE ( 'NONE', #98960, 0.1000000000000000472, 0.003490658503988666988 ) ;
#111475=ORIENTED_EDGE ( 'NONE', *, *, #42626, .T. ) ;
#111476=DIRECTION ( 'NONE',  ( -0.000000000000000000, -1.000000000000000000, -0.000000000000000000 ) ) ;
#111477=CONICAL_SURFACE ( 'NONE', #105218, 0.09999999999999982514, 0.003490658503988666988 ) ;
#111478=ORIENTED_EDGE ( 'NONE', *, *, #112042, .F. ) ;
#111479=DIRECTION ( 'NONE',  ( 0.000000000000000000, 0.000000000000000000, 1.000000000000000000 ) ) ;
#111480=AXIS2_PLACEMENT_3D ( 'NONE', #120942, #113052, #24047 ) ;
#111481=EDGE_LOOP ( 'NONE', ( #68592, #101082 ) ) ;
#111482=CONICAL_SURFACE ( 'NONE', #88488, 0.1000000000000002554, 0.003490658503988666988 ) ;
#111483=LINE ( 'NONE', #101678, #67702 ) ;
#111484=ORIENTED_EDGE ( 'NONE', *, *, #56071, .F. ) ;
#111485=VECTOR ( 'NONE', #8600, 1000.000000000000000 ) ;
#111486=FACE_OUTER_BOUND ( 'NONE', #63844, .T. ) ;
#111487=DIRECTION ( 'NONE',  ( 0.000000000000000000, -0.000000000000000000, 1.000000000000000000 ) ) ;
#111488=ORIENTED_EDGE ( 'NONE', *, *, #80176, .F. ) ;
#111489=ORIENTED_EDGE ( 'NONE', *, *, #35976, .F. ) ;
#111490=DIRECTION ( 'NONE',  ( 0.000000000000000000, 0.000000000000000000, -1.000000000000000000 ) ) ;
#111491=DIRECTION ( 'NONE',  ( -4.274815082592931898E-19, -0.9999939076577903929, -0.003490651415223739937 ) ) ;
#111492=DIRECTION ( 'NONE',  ( -4.274815082592931898E-19, -0.9999939076577903929, -0.003490651415223739937 ) ) ;
#111493=CARTESIAN_POINT ( 'NONE',  ( 1.449999999999952216, 2.500000000000000000, 1.818653347947321475 ) ) ;
#111494=AXIS2_PLACEMENT_3D ( 'NONE', #127173, #27642, #25725 ) ;
#111495=PLANE ( 'NONE',  #16579 ) ;
#111496=ORIENTED_EDGE ( 'NONE', *, *, #7593, .T. ) ;
#111497=DIRECTION ( 'NONE',  ( 0.000000000000000000, 0.000000000000000000, 1.000000000000000000 ) ) ;
#111498=EDGE_CURVE ( 'NONE', #100972, #113211, #20318, .T. ) ;
#111499=EDGE_CURVE ( 'NONE', #90496, #36406, #76564, .T. ) ;
#111500=AXIS2_PLACEMENT_3D ( 'NONE', #122327, #120385, #110552 ) ;
#111501=ADVANCED_FACE ( 'NONE', ( #6552 ), #32677, .T. ) ;
#111502=ORIENTED_EDGE ( 'NONE', *, *, #58771, .T. ) ;
#111503=AXIS2_PLACEMENT_3D ( 'NONE', #82772, #53305, #101102 ) ;
#111504=DIRECTION ( 'NONE',  ( -0.000000000000000000, -1.000000000000000000, -0.000000000000000000 ) ) ;
#111505=DIRECTION ( 'NONE',  ( 0.000000000000000000, -0.9999939076577903929, 0.003490651415223739937 ) ) ;
#111506=AXIS2_PLACEMENT_3D ( 'NONE', #57947, #128639, #107012 ) ;
#111507=EDGE_CURVE ( 'NONE', #52727, #17050, #36778, .T. ) ;
#111509=CARTESIAN_POINT ( 'NONE',  ( -12.09999999999999432, 12.50000000000000000, 3.572213422710607489 ) ) ;
#111510=CARTESIAN_POINT ( 'NONE',  ( -9.150000000000009237, 12.50000000000000000, 2.922977105672686982 ) ) ;
#111511=EDGE_CURVE ( 'NONE', #39415, #13047, #30525, .T. ) ;
#111512=DIRECTION ( 'NONE',  ( 0.000000000000000000, 0.000000000000000000, 1.000000000000000000 ) ) ;
#111513=AXIS2_PLACEMENT_3D ( 'NONE', #126858, #57475, #105925 ) ;
#111514=CARTESIAN_POINT ( 'NONE',  ( -10.40000000000000213, 2.500000000000000000, 4.430127018922196847 ) ) ;
#111515=AXIS2_PLACEMENT_3D ( 'NONE', #39066, #129382, #8915 ) ;
#111516=EDGE_LOOP ( 'NONE', ( #55261, #57659, #94112, #89405 ) ) ;
#111517=ADVANCED_FACE ( 'NONE', ( #108013 ), #25574, .T. ) ;
#111519=EDGE_CURVE ( 'NONE', #115994, #5036, #101606, .T. ) ;
#111520=AXIS2_PLACEMENT_3D ( 'NONE', #98616, #18137, #108450 ) ;
#111521=CARTESIAN_POINT ( 'NONE',  ( 7.049999999999926992, 2.500000000000000000, 2.265063509461097357 ) ) ;
#111522=EDGE_CURVE ( 'NONE', #54526, #2989, #9659, .T. ) ;
#111523=CARTESIAN_POINT ( 'NONE',  ( -3.100000000000028511, 2.500000000000000000, -0.2464101615137782308 ) ) ;
#111524=DIRECTION ( 'NONE',  ( 0.000000000000000000, 0.000000000000000000, 1.000000000000000000 ) ) ;
#111525=AXIS2_PLACEMENT_3D ( 'NONE', #53488, #3098, #15 ) ;
#111526=EDGE_LOOP ( 'NONE', ( #68191, #5941, #66069, #8578 ) ) ;
#111527=EDGE_CURVE ( 'NONE', #91651, #224, #70208, .T. ) ;
#111528=FACE_OUTER_BOUND ( 'NONE', #10661, .T. ) ;
#111529=ORIENTED_EDGE ( 'NONE', *, *, #45187, .T. ) ;
#111530=VECTOR ( 'NONE', #9477, 1000.000000000000000 ) ;
#111531=AXIS2_PLACEMENT_3D ( 'NONE', #58540, #17950, #19897 ) ;
#111533=AXIS2_PLACEMENT_3D ( 'NONE', #84885, #53507, #113051 ) ;
#111534=DIRECTION ( 'NONE',  ( 0.000000000000000000, 0.000000000000000000, 1.000000000000000000 ) ) ;
#111535=AXIS2_PLACEMENT_3D ( 'NONE', #86770, #67104, #37049 ) ;
#111536=ORIENTED_EDGE ( 'NONE', *, *, #21602, .T. ) ;
#111537=CARTESIAN_POINT ( 'NONE',  ( 18.93069778776242273, -2.571126379696489828, -2.451182541063237075 ) ) ;
#111538=CARTESIAN_POINT ( 'NONE',  ( 0.4499999999999552136, 2.500000000000000000, 6.495190528383297135 ) ) ;
#111539=CARTESIAN_POINT ( 'NONE',  ( 20.06694580393655158, 2.635910463901408374, 2.269534205244102321 ) ) ;
#111540=VECTOR ( 'NONE', #68894, 1000.000000000000000 ) ;
#111541=EDGE_LOOP ( 'NONE', ( #120696, #128432, #93745, #31304 ) ) ;
#111542=DIRECTION ( 'NONE',  ( 0.000000000000000000, 1.000000000000000000, 0.000000000000000000 ) ) ;
#111543=CARTESIAN_POINT ( 'NONE',  ( 5.399999999999935518, 12.50000000000000000, -4.330127018922201643 ) ) ;
#111544=EDGE_CURVE ( 'NONE', #46534, #3135, #36716, .T. ) ;
#111545=ORIENTED_EDGE ( 'NONE', *, *, #73933, .T. ) ;
#111546=ORIENTED_EDGE ( 'NONE', *, *, #34554, .F. ) ;
#111547=VERTEX_POINT ( 'NONE', #26246 ) ;
#111548=DIRECTION ( 'NONE',  ( -0.000000000000000000, 1.000000000000000000, -0.000000000000000000 ) ) ;
#111549=DIRECTION ( 'NONE',  ( 0.000000000000000000, 1.000000000000000000, 0.000000000000000000 ) ) ;
#111550=AXIS2_PLACEMENT_3D ( 'NONE', #43724, #4384, #44333 ) ;
#111551=CARTESIAN_POINT ( 'NONE',  ( 13.54999999999989946, 12.50000000000000000, 2.511473670974873507 ) ) ;
#111552=FACE_BOUND ( 'NONE', #69228, .T. ) ;
#111553=ORIENTED_EDGE ( 'NONE', *, *, #35668, .F. ) ;
#111554=CARTESIAN_POINT ( 'NONE',  ( -1.900000000000034550, 2.500000000000000000, 4.776537180435972196 ) ) ;
#111555=FACE_OUTER_BOUND ( 'NONE', #122859, .T. ) ;
#111556=EDGE_LOOP ( 'NONE', ( #30171, #94767 ) ) ;
#111557=DIRECTION ( 'NONE',  ( 0.000000000000000000, 1.000000000000000000, 0.000000000000000000 ) ) ;
#111558=CARTESIAN_POINT ( 'NONE',  ( 5.399999999999932854, 2.500000000000000000, 5.022947341949748790 ) ) ;
#111559=AXIS2_PLACEMENT_3D ( 'NONE', #27285, #107131, #97963 ) ;
#111560=ADVANCED_FACE ( 'NONE', ( #56327 ), #49392, .T. ) ;
#111561=CONICAL_SURFACE ( 'NONE', #105208, 0.1000000000000000472, 0.003490658503988666988 ) ;
#111562=CONICAL_SURFACE ( 'NONE', #32169, 0.1000000000000002554, 0.003490658503988666988 ) ;
#111563=DIRECTION ( 'NONE',  ( 0.000000000000000000, 0.000000000000000000, 1.000000000000000000 ) ) ;
#111564=CIRCLE ( 'NONE', #103154, 0.1000000000000002554 ) ;
#111565=DIRECTION ( 'NONE',  ( -4.274815082592931898E-19, -0.9999939076577903929, -0.003490651415223739937 ) ) ;
#111566=CARTESIAN_POINT ( 'NONE',  ( 12.09999999999990550, 2.500000000000000000, -3.737306695894649700 ) ) ;
#111567=CARTESIAN_POINT ( 'NONE',  ( -0.4500000000000397571, 2.500000000000000000, -6.495190528383302464 ) ) ;
#111568=DIRECTION ( 'NONE',  ( 0.000000000000000000, -0.000000000000000000, 1.000000000000000000 ) ) ;
#111569=CONICAL_SURFACE ( 'NONE', #88588, 0.1000000000000002554, 0.003490658503988666988 ) ;
#111570=CIRCLE ( 'NONE', #67745, 0.1000000000000002554 ) ;
#111571=CIRCLE ( 'NONE', #32180, 0.06509327318403745899 ) ;
#111572=ORIENTED_EDGE ( 'NONE', *, *, #26639, .F. ) ;
#111573=VERTEX_POINT ( 'NONE', #45886 ) ;
#111574=ORIENTED_EDGE ( 'NONE', *, *, #41468, .T. ) ;
#111575=VERTEX_POINT ( 'NONE', #77272 ) ;
#111576=DIRECTION ( 'NONE',  ( -0.000000000000000000, -1.000000000000000000, -0.000000000000000000 ) ) ;
#111577=CIRCLE ( 'NONE', #76170, 0.06509327318403745899 ) ;
#111578=CARTESIAN_POINT ( 'NONE',  ( 5.799999999999931433, 2.500000000000000000, 4.430127018922196847 ) ) ;
#111579=ORIENTED_EDGE ( 'NONE', *, *, #56745, .T. ) ;
#111580=EDGE_CURVE ( 'NONE', #125708, #120954, #8510, .T. ) ;
#111581=FACE_BOUND ( 'NONE', #72039, .T. ) ;
#111583=CARTESIAN_POINT ( 'NONE',  ( 0.4499999999999569344, 12.50000000000000000, -2.165063509461101710 ) ) ;
#111584=DIRECTION ( 'NONE',  ( -4.274815082592931898E-19, -0.9999939076577903929, -0.003490651415223739937 ) ) ;
#111585=DIRECTION ( 'NONE',  ( 0.000000000000000000, 0.000000000000000000, 1.000000000000000000 ) ) ;
#111586=DIRECTION ( 'NONE',  ( -0.000000000000000000, 1.000000000000000000, -0.000000000000000000 ) ) ;
#111587=LINE ( 'NONE', #118827, #101873 ) ;
#111588=DIRECTION ( 'NONE',  ( 0.000000000000000000, -0.000000000000000000, 1.000000000000000000 ) ) ;
#111589=CARTESIAN_POINT ( 'NONE',  ( -11.89999999999999680, 12.50000000000000000, 0.3464101615137776813 ) ) ;
#111591=DIRECTION ( 'NONE',  ( 0.000000000000000000, 0.000000000000000000, -1.000000000000000000 ) ) ;
#111592=EDGE_LOOP ( 'NONE', ( #79483, #64185 ) ) ;
#111593=AXIS2_PLACEMENT_3D ( 'NONE', #53748, #124429, #42666 ) ;
#111594=EDGE_LOOP ( 'NONE', ( #77815, #23027 ) ) ;
#111595=VERTEX_POINT ( 'NONE', #55691 ) ;
#111596=EDGE_LOOP ( 'NONE', ( #34255, #118721, #68364, #74566 ) ) ;
#111597=EDGE_LOOP ( 'NONE', ( #78445, #1485 ) ) ;
#111598=VERTEX_POINT ( 'NONE', #57639 ) ;
#111599=CARTESIAN_POINT ( 'NONE',  ( 3.349999999999944578, 2.500000000000000000, -1.372243186433550033 ) ) ;
#111600=EDGE_LOOP ( 'NONE', ( #41498, #7388, #45423, #118198 ) ) ;
#111601=EDGE_LOOP ( 'NONE', ( #38846, #485, #106599, #68152 ) ) ;
#111602=CIRCLE ( 'NONE', #86450, 0.06509327318403745899 ) ;
#111603=AXIS2_PLACEMENT_3D ( 'NONE', #806, #80673, #42031 ) ;
#111604=AXIS2_PLACEMENT_3D ( 'NONE', #34123, #32204, #53752 ) ;
#111606=DIRECTION ( 'NONE',  ( 0.000000000000000000, 0.000000000000000000, 1.000000000000000000 ) ) ;
#111607=CARTESIAN_POINT ( 'NONE',  ( -11.89999999999999503, 12.50000000000000000, 4.676537180435972552 ) ) ;
#111608=CARTESIAN_POINT ( 'NONE',  ( 6.649999999999930189, 2.500000000000000000, 5.802370205355744659 ) ) ;
#111609=DIRECTION ( 'NONE',  ( -0.000000000000000000, -1.000000000000000000, -0.000000000000000000 ) ) ;
#111610=AXIS2_PLACEMENT_3D ( 'NONE', #41708, #22070, #12217 ) ;
#111611=ORIENTED_EDGE ( 'NONE', *, *, #14775, .F. ) ;
#111612=DIRECTION ( 'NONE',  ( 0.000000000000000000, 0.000000000000000000, 1.000000000000000000 ) ) ;
#111613=AXIS2_PLACEMENT_3D ( 'NONE', #82849, #1676, #62560 ) ;
#111614=AXIS2_PLACEMENT_3D ( 'NONE', #114191, #55274, #125298 ) ;
#111615=EDGE_LOOP ( 'NONE', ( #18614, #21918, #75614, #93717 ) ) ;
#111616=VECTOR ( 'NONE', #101868, 1000.000000000000000 ) ;
#111617=VERTEX_POINT ( 'NONE', #75978 ) ;
#111618=DIRECTION ( 'NONE',  ( -4.274815082592931898E-19, -0.9999939076577903929, -0.003490651415223739937 ) ) ;
#111620=DIRECTION ( 'NONE',  ( 0.000000000000000000, 0.000000000000000000, 1.000000000000000000 ) ) ;
#111621=FACE_OUTER_BOUND ( 'NONE', #118891, .T. ) ;
#111622=EDGE_CURVE ( 'NONE', #88783, #13760, #114118, .T. ) ;
#111623=EDGE_CURVE ( 'NONE', #61624, #83259, #55634, .T. ) ;
#111624=EDGE_CURVE ( 'NONE', #73740, #16607, #95128, .T. ) ;
#111625=VERTEX_POINT ( 'NONE', #41237 ) ;
#111626=ORIENTED_EDGE ( 'NONE', *, *, #34966, .F. ) ;
#111627=DIRECTION ( 'NONE',  ( -0.000000000000000000, 1.000000000000000000, -0.000000000000000000 ) ) ;
#111628=DIRECTION ( 'NONE',  ( 0.000000000000000000, 1.000000000000000000, 0.000000000000000000 ) ) ;
#111629=CIRCLE ( 'NONE', #51005, 0.09999999999999982514 ) ;
#111630=EDGE_CURVE ( 'NONE', #62406, #64648, #20047, .T. ) ;
#111631=DIRECTION ( 'NONE',  ( 0.000000000000000000, -0.000000000000000000, 1.000000000000000000 ) ) ;
#111632=CIRCLE ( 'NONE', #7052, 0.1000000000000002554 ) ;
#111633=CONICAL_SURFACE ( 'NONE', #13414, 0.1000000000000002554, 0.003490658503988666988 ) ;
#111634=CARTESIAN_POINT ( 'NONE',  ( 1.649999999999950617, 12.50000000000000000, -2.165063509461101710 ) ) ;
#111635=PLANE ( 'NONE',  #75312 ) ;
#111636=CIRCLE ( 'NONE', #46888, 0.09999999999999982514 ) ;
#111637=EDGE_CURVE ( 'NONE', #75483, #24362, #93203, .T. ) ;
#111638=ORIENTED_EDGE ( 'NONE', *, *, #115485, .F. ) ;
#111639=CIRCLE ( 'NONE', #86581, 0.09999999999999982514 ) ;
#111640=CARTESIAN_POINT ( 'NONE',  ( -14.59999999999998366, 2.500000000000000000, 0.6928203230275518099 ) ) ;
#111641=EDGE_CURVE ( 'NONE', #101677, #91963, #11710, .T. ) ;
#111642=EDGE_CURVE ( 'NONE', #84952, #120463, #26399, .T. ) ;
#111643=EDGE_LOOP ( 'NONE', ( #117549, #78846 ) ) ;
#111644=CARTESIAN_POINT ( 'NONE',  ( 87.50000000000002842, 4.871203238224194543, -5.733266569811712010 ) ) ;
#111645=CARTESIAN_POINT ( 'NONE',  ( 2.499999999999947153, 12.50000000000000000, -3.572213422710612374 ) ) ;
#111646=PLANE ( 'NONE',  #34403 ) ;
#111647=DIRECTION ( 'NONE',  ( 0.000000000000000000, 0.000000000000000000, -1.000000000000000000 ) ) ;
#111649=DIRECTION ( 'NONE',  ( 0.000000000000000000, -0.9999939076577903929, 0.003490651415223739937 ) ) ;
#111650=ADVANCED_FACE ( 'NONE', ( #18982 ), #128822, .T. ) ;
#111651=EDGE_LOOP ( 'NONE', ( #101377, #18783 ) ) ;
#111652=DIRECTION ( 'NONE',  ( 0.000000000000000000, 1.000000000000000000, 0.000000000000000000 ) ) ;
#111653=CIRCLE ( 'NONE', #36455, 0.06509327318403745899 ) ;
#111654=DIRECTION ( 'NONE',  ( 0.000000000000000000, 0.000000000000000000, 1.000000000000000000 ) ) ;
#111655=VERTEX_POINT ( 'NONE', #58924 ) ;
#111656=VERTEX_POINT ( 'NONE', #81150 ) ;
#111657=AXIS2_PLACEMENT_3D ( 'NONE', #67276, #106591, #107238 ) ;
#111658=ORIENTED_EDGE ( 'NONE', *, *, #28487, .F. ) ;
#111659=CARTESIAN_POINT ( 'NONE',  ( 17.50000000000000000, 0.9166666666666682950, 4.000000000000001776 ) ) ;
#111660=DIRECTION ( 'NONE',  ( -0.000000000000000000, -1.000000000000000000, -0.000000000000000000 ) ) ;
#111661=DIRECTION ( 'NONE',  ( 0.000000000000000000, 0.000000000000000000, 1.000000000000000000 ) ) ;
#111662=LINE ( 'NONE', #22009, #63721 ) ;
#111663=DIRECTION ( 'NONE',  ( -0.000000000000000000, -1.000000000000000000, -0.000000000000000000 ) ) ;
#111664=VECTOR ( 'NONE', #66923, 1000.000000000000000 ) ;
#111665=AXIS2_PLACEMENT_3D ( 'NONE', #53392, #12156, #92019 ) ;
#111666=FACE_OUTER_BOUND ( 'NONE', #117114, .T. ) ;
#111667=AXIS2_PLACEMENT_3D ( 'NONE', #20564, #81424, #101050 ) ;
#111668=DIRECTION ( 'NONE',  ( -4.274815082592931898E-19, -0.9999939076577903929, -0.003490651415223739937 ) ) ;
#111670=CIRCLE ( 'NONE', #46825, 0.06509327318403745899 ) ;
#111671=EDGE_CURVE ( 'NONE', #75028, #34064, #70038, .T. ) ;
#111672=CONICAL_SURFACE ( 'NONE', #57287, 0.09999999999999982514, 0.003490658503988666988 ) ;
#111673=AXIS2_PLACEMENT_3D ( 'NONE', #30689, #120983, #41803 ) ;
#111674=ORIENTED_EDGE ( 'NONE', *, *, #45501, .F. ) ;
#111675=FACE_OUTER_BOUND ( 'NONE', #88312, .T. ) ;
#111676=CONICAL_SURFACE ( 'NONE', #97001, 0.09999999999999982514, 0.003490658503988666988 ) ;
#111677=DIRECTION ( 'NONE',  ( 0.000000000000000000, -0.000000000000000000, 1.000000000000000000 ) ) ;
#111678=FACE_OUTER_BOUND ( 'NONE', #8161, .T. ) ;
#111679=DIRECTION ( 'NONE',  ( 0.000000000000000000, 0.000000000000000000, -1.000000000000000000 ) ) ;
#111680=EDGE_LOOP ( 'NONE', ( #27900, #26726, #111966, #71975 ) ) ;
#111681=CARTESIAN_POINT ( 'NONE',  ( -13.74999999999998934, 2.500000000000000000, -1.472243186433547901 ) ) ;
#111682=EDGE_CURVE ( 'NONE', #15887, #109919, #57699, .T. ) ;
#111683=EDGE_CURVE ( 'NONE', #122356, #36724, #51692, .T. ) ;
#111684=DIRECTION ( 'NONE',  ( 0.000000000000000000, 0.000000000000000000, 1.000000000000000000 ) ) ;
#111685=CARTESIAN_POINT ( 'NONE',  ( 8.299999999999922551, 12.50000000000000000, -4.330127018922201643 ) ) ;
#111686=ORIENTED_EDGE ( 'NONE', *, *, #65718, .T. ) ;
#111687=CIRCLE ( 'NONE', #128437, 0.06509327318403745899 ) ;
#111688=ORIENTED_EDGE ( 'NONE', *, *, #42177, .F. ) ;
#111689=EDGE_CURVE ( 'NONE', #62384, #14824, #24242, .T. ) ;
#111690=DIRECTION ( 'NONE',  ( 0.000000000000000000, -0.000000000000000000, 1.000000000000000000 ) ) ;
#111691=ORIENTED_EDGE ( 'NONE', *, *, #112002, .T. ) ;
#111692=EDGE_LOOP ( 'NONE', ( #110589, #108009, #33941, #94653 ) ) ;
#111693=DIRECTION ( 'NONE',  ( 0.000000000000000000, 0.000000000000000000, 1.000000000000000000 ) ) ;
#111694=FACE_OUTER_BOUND ( 'NONE', #121443, .T. ) ;
#111696=AXIS2_PLACEMENT_3D ( 'NONE', #22738, #43032, #113023 ) ;
#111697=CARTESIAN_POINT ( 'NONE',  ( 13.14999999999989733, 2.500000000000000000, -2.511473670974877948 ) ) ;
#111698=CONICAL_SURFACE ( 'NONE', #51165, 0.1000000000000000472, 0.003490658503988666988 ) ;
#111699=EDGE_LOOP ( 'NONE', ( #12533, #9909, #78018, #88770 ) ) ;
#111700=DIRECTION ( 'NONE',  ( 0.000000000000000000, 1.000000000000000000, 0.000000000000000000 ) ) ;
#111701=ORIENTED_EDGE ( 'NONE', *, *, #83718, .F. ) ;
#111702=CARTESIAN_POINT ( 'NONE',  ( -3.950000000000029932, 2.500000000000000000, -6.148780366869526226 ) ) ;
#111703=FACE_OUTER_BOUND ( 'NONE', #66838, .T. ) ;
#111704=VERTEX_POINT ( 'NONE', #633 ) ;
#111705=AXIS2_PLACEMENT_3D ( 'NONE', #41528, #70961, #99139 ) ;
#111706=EDGE_LOOP ( 'NONE', ( #122200, #81143, #52094, #115989 ) ) ;
#111707=ORIENTED_EDGE ( 'NONE', *, *, #82069, .T. ) ;
#111708=ORIENTED_EDGE ( 'NONE', *, *, #104846, .T. ) ;
#111709=CARTESIAN_POINT ( 'NONE',  ( -1.650000000000035660, 2.500000000000000000, 2.957883832488649389 ) ) ;
#111710=LINE ( 'NONE', #20110, #35314 ) ;
#111711=DIRECTION ( 'NONE',  ( 0.000000000000000000, 0.000000000000000000, 1.000000000000000000 ) ) ;
#111712=FACE_BOUND ( 'NONE', #23293, .T. ) ;
#111713=ORIENTED_EDGE ( 'NONE', *, *, #43289, .F. ) ;
#111714=DIRECTION ( 'NONE',  ( 0.000000000000000000, -0.9999939076577903929, 0.003490651415223739937 ) ) ;
#111716=CARTESIAN_POINT ( 'NONE',  ( 8.549999999999922551, 12.50000000000000000, -6.213873640053564351 ) ) ;
#111717=CARTESIAN_POINT ( 'NONE',  ( -1.250000000000001110, 12.50000000000000000, -6.495190528383302464 ) ) ;
#111718=CIRCLE ( 'NONE', #94998, 0.06509327318403745899 ) ;
#111719=DIRECTION ( 'NONE',  ( 0.000000000000000000, 0.000000000000000000, 1.000000000000000000 ) ) ;
#111720=CARTESIAN_POINT ( 'NONE',  ( -11.89999999999999680, 2.500000000000000000, -3.983716857408423628 ) ) ;
#111721=DIRECTION ( 'NONE',  ( 0.000000000000000000, -0.9999939076577903929, 0.003490651415223739937 ) ) ;
#111722=CONICAL_SURFACE ( 'NONE', #122198, 0.09999999999999982514, 0.003490658503988666988 ) ;
#111723=CARTESIAN_POINT ( 'NONE',  ( 11.24999999999991118, 12.50000000000000000, 5.867463478539781896 ) ) ;
#111724=ORIENTED_EDGE ( 'NONE', *, *, #126904, .T. ) ;
#111725=ORIENTED_EDGE ( 'NONE', *, *, #105236, .T. ) ;
#111726=ORIENTED_EDGE ( 'NONE', *, *, #63155, .T. ) ;
#111727=ORIENTED_EDGE ( 'NONE', *, *, #73991, .F. ) ;
#111728=EDGE_CURVE ( 'NONE', #65690, #7809, #99560, .T. ) ;
#111729=ORIENTED_EDGE ( 'NONE', *, *, #22573, .T. ) ;
#111730=DIRECTION ( 'NONE',  ( 0.000000000000000000, 0.000000000000000000, 1.000000000000000000 ) ) ;
#111731=FACE_OUTER_BOUND ( 'NONE', #80618, .T. ) ;
#111732=ORIENTED_EDGE ( 'NONE', *, *, #53993, .T. ) ;
#111733=EDGE_CURVE ( 'NONE', #20397, #14404, #9821, .T. ) ;
#111734=FACE_BOUND ( 'NONE', #18432, .T. ) ;
#111735=CARTESIAN_POINT ( 'NONE',  ( 8.349999999999923261, 2.500000000000000000, -7.188010851410854052 ) ) ;
#111736=AXIS2_PLACEMENT_3D ( 'NONE', #44508, #43888, #84439 ) ;
#111737=AXIS2_PLACEMENT_3D ( 'NONE', #29245, #109728, #69798 ) ;
#111738=VERTEX_POINT ( 'NONE', #10459 ) ;
#111739=FACE_OUTER_BOUND ( 'NONE', #125656, .T. ) ;
#111740=VECTOR ( 'NONE', #89391, 1000.000000000000000 ) ;
#111741=CARTESIAN_POINT ( 'NONE',  ( -12.49999999999999467, 2.500000000000000000, 0.5928203230275536084 ) ) ;
#111742=EDGE_CURVE ( 'NONE', #56826, #33171, #59868, .T. ) ;
#111743=DIRECTION ( 'NONE',  ( -0.000000000000000000, 1.000000000000000000, -0.000000000000000000 ) ) ;
#111744=CARTESIAN_POINT ( 'NONE',  ( -8.350000000000012079, 12.50000000000000000, -2.857883832488653741 ) ) ;
#111745=ORIENTED_EDGE ( 'NONE', *, *, #56839, .F. ) ;
#111746=DIRECTION ( 'NONE',  ( 0.000000000000000000, 1.000000000000000000, 0.000000000000000000 ) ) ;
#111747=VECTOR ( 'NONE', #22788, 1000.000000000000000 ) ;
#111748=ORIENTED_EDGE ( 'NONE', *, *, #71402, .T. ) ;
#111749=AXIS2_PLACEMENT_3D ( 'NONE', #86469, #55727, #116570 ) ;
#111750=VECTOR ( 'NONE', #34263, 1000.000000000000000 ) ;
#111751=ORIENTED_EDGE ( 'NONE', *, *, #73766, .T. ) ;
#111752=EDGE_LOOP ( 'NONE', ( #17279, #88034, #113476, #7846 ) ) ;
#111753=CARTESIAN_POINT ( 'NONE',  ( 2.899999999999945732, 12.50000000000000000, -4.395220292106239768 ) ) ;
#111754=AXIS2_PLACEMENT_3D ( 'NONE', #126322, #28775, #107318 ) ;
#111755=DIRECTION ( 'NONE',  ( -0.000000000000000000, 1.000000000000000000, -0.000000000000000000 ) ) ;
#111756=EDGE_LOOP ( 'NONE', ( #38450, #75014, #48800, #49348 ) ) ;
#111757=DIRECTION ( 'NONE',  ( -0.000000000000000000, 1.000000000000000000, -0.000000000000000000 ) ) ;
#111758=AXIS2_PLACEMENT_3D ( 'NONE', #109881, #60154, #82366 ) ;
#111759=CIRCLE ( 'NONE', #86715, 2.000000000000000000 ) ;
#111760=CARTESIAN_POINT ( 'NONE',  ( 0.000000000000000000, 12.50000000000000000, 0.000000000000000000 ) ) ;
#111761=DIRECTION ( 'NONE',  ( 0.000000000000000000, 0.000000000000000000, 1.000000000000000000 ) ) ;
#111762=EDGE_CURVE ( 'NONE', #51026, #71846, #11752, .T. ) ;
#111763=DIRECTION ( 'NONE',  ( -0.000000000000000000, -1.000000000000000000, -0.000000000000000000 ) ) ;
#111765=CIRCLE ( 'NONE', #86717, 0.06509327318403745899 ) ;
#111766=VERTEX_POINT ( 'NONE', #39940 ) ;
#111767=FACE_OUTER_BOUND ( 'NONE', #77885, .T. ) ;
#111768=ORIENTED_EDGE ( 'NONE', *, *, #63280, .F. ) ;
#111769=CARTESIAN_POINT ( 'NONE',  ( -4.400000000000025224, 12.50000000000000000, 3.983716857408420076 ) ) ;
#111770=EDGE_CURVE ( 'NONE', #31773, #120101, #1253, .T. ) ;
#111771=ORIENTED_EDGE ( 'NONE', *, *, #118745, .F. ) ;
#111772=CARTESIAN_POINT ( 'NONE',  ( -9.400000000000007461, 2.500000000000000000, 4.576537180435972019 ) ) ;
#111773=EDGE_LOOP ( 'NONE', ( #14796, #3552 ) ) ;
#111774=CARTESIAN_POINT ( 'NONE',  ( -8.150000000000012790, 2.500000000000000000, 1.818653347947321475 ) ) ;
#111775=DIRECTION ( 'NONE',  ( -0.000000000000000000, 1.000000000000000000, -0.000000000000000000 ) ) ;
#111776=EDGE_CURVE ( 'NONE', #78026, #116101, #78640, .T. ) ;
#111777=DIRECTION ( 'NONE',  ( 0.000000000000000000, 0.000000000000000000, -1.000000000000000000 ) ) ;
#111778=CARTESIAN_POINT ( 'NONE',  ( -5.600000000000023626, 2.500000000000000000, -3.883716857408426648 ) ) ;
#111779=ADVANCED_FACE ( 'NONE', ( #100757 ), #24157, .T. ) ;
#111780=EDGE_CURVE ( 'NONE', #20674, #97708, #32060, .T. ) ;
#111781=FACE_OUTER_BOUND ( 'NONE', #120930, .T. ) ;
#111782=EDGE_CURVE ( 'NONE', #60985, #49812, #22202, .T. ) ;
#111783=VECTOR ( 'NONE', #59354, 1000.000000000000000 ) ;
#111784=ORIENTED_EDGE ( 'NONE', *, *, #90940, .F. ) ;
#111785=ORIENTED_EDGE ( 'NONE', *, *, #102423, .F. ) ;
#111786=FACE_OUTER_BOUND ( 'NONE', #39182, .T. ) ;
#111787=CARTESIAN_POINT ( 'NONE',  ( 3.299999999999944755, 12.50000000000000000, -2.385244779468109755E-15 ) ) ;
#111788=EDGE_CURVE ( 'NONE', #121167, #127574, #71980, .T. ) ;
#111789=CARTESIAN_POINT ( 'NONE',  ( 6.649999999999930189, 2.500000000000000000, -2.857883832488653741 ) ) ;
#111790=ORIENTED_EDGE ( 'NONE', *, *, #106328, .F. ) ;
#111791=EDGE_LOOP ( 'NONE', ( #47040, #26100 ) ) ;
#111792=ORIENTED_EDGE ( 'NONE', *, *, #101028, .F. ) ;
#111793=ADVANCED_FACE ( 'NONE', ( #13673 ), #61994, .T. ) ;
#111794=LINE ( 'NONE', #21472, #93785 ) ;
#111795=ORIENTED_EDGE ( 'NONE', *, *, #39862, .T. ) ;
#111796=DIRECTION ( 'NONE',  ( -0.000000000000000000, -1.000000000000000000, -0.000000000000000000 ) ) ;
#111797=DIRECTION ( 'NONE',  ( 0.000000000000000000, -0.000000000000000000, 1.000000000000000000 ) ) ;
#111798=CONICAL_SURFACE ( 'NONE', #88800, 0.1000000000000002554, 0.003490658503988666988 ) ;
#111799=EDGE_CURVE ( 'NONE', #87462, #105143, #89089, .T. ) ;
#111801=EDGE_CURVE ( 'NONE', #114386, #49349, #49485, .T. ) ;
#111803=ORIENTED_EDGE ( 'NONE', *, *, #104290, .T. ) ;
#111804=CARTESIAN_POINT ( 'NONE',  ( -10.00000000000000533, 2.500000000000000000, -5.122947341949750211 ) ) ;
#111805=DIRECTION ( 'NONE',  ( 0.000000000000000000, -0.9999939076577903929, 0.003490651415223739937 ) ) ;
#111806=CARTESIAN_POINT ( 'NONE',  ( -4.550000000000026468, 2.500000000000000000, -6.395190528383301931 ) ) ;
#111807=CARTESIAN_POINT ( 'NONE',  ( 1.049999999999954969, 2.500000000000000000, -6.941600689897077459 ) ) ;
#111808=DIRECTION ( 'NONE',  ( 0.000000000000000000, 0.000000000000000000, 1.000000000000000000 ) ) ;
#111809=EDGE_CURVE ( 'NONE', #8589, #25026, #2552, .T. ) ;
#111810=EDGE_LOOP ( 'NONE', ( #29747, #27735 ) ) ;
#111811=AXIS2_PLACEMENT_3D ( 'NONE', #108145, #27634, #67565 ) ;
#111812=CARTESIAN_POINT ( 'NONE',  ( -1.224646799147353269E-17, 2.500000000000000000, -0.1000000000000000056 ) ) ;
#111813=CARTESIAN_POINT ( 'NONE',  ( 1.649999999999950617, 12.50000000000000000, 2.099970236277060032 ) ) ;
#111814=CIRCLE ( 'NONE', #80705, 0.06509327318403745899 ) ;
#111815=ORIENTED_EDGE ( 'NONE', *, *, #38212, .F. ) ;
#111816=ORIENTED_EDGE ( 'NONE', *, *, #29479, .F. ) ;
#111818=PLANE ( 'NONE',  #34416 ) ;
#111819=CARTESIAN_POINT ( 'NONE',  ( -7.100000000000017408, 2.500000000000000000, -3.737306695894649700 ) ) ;
#111820=DIRECTION ( 'NONE',  ( -0.000000000000000000, 1.000000000000000000, -0.000000000000000000 ) ) ;
#111821=DIRECTION ( 'NONE',  ( -0.000000000000000000, -1.000000000000000000, -0.000000000000000000 ) ) ;
#111822=CARTESIAN_POINT ( 'NONE',  ( 0.8499999999999553468, 12.50000000000000000, 2.099970236277060032 ) ) ;
#111823=CONICAL_SURFACE ( 'NONE', #44920, 0.09999999999999982514, 0.003490658503988666988 ) ;
#111824=DIRECTION ( 'NONE',  ( 0.000000000000000000, 1.000000000000000000, 0.000000000000000000 ) ) ;
#111825=CARTESIAN_POINT ( 'NONE',  ( -14.59999999999998366, 12.50000000000000000, -1.084202172485504434E-16 ) ) ;
#111826=CIRCLE ( 'NONE', #34180, 0.06509327318403745899 ) ;
#111827=AXIS2_PLACEMENT_3D ( 'NONE', #61832, #110268, #81463 ) ;
#111828=DIRECTION ( 'NONE',  ( 0.000000000000000000, 1.000000000000000000, 0.000000000000000000 ) ) ;
#111829=ORIENTED_EDGE ( 'NONE', *, *, #84010, .F. ) ;
#111830=VERTEX_POINT ( 'NONE', #41876 ) ;
#111831=VERTEX_POINT ( 'NONE', #1922 ) ;
#111832=ORIENTED_EDGE ( 'NONE', *, *, #16590, .T. ) ;
#111833=CARTESIAN_POINT ( 'NONE',  ( -6.250000000000015987, 2.500000000000000000, 5.902370205355745192 ) ) ;
#111834=DIRECTION ( 'NONE',  ( 0.000000000000000000, 1.000000000000000000, 0.000000000000000000 ) ) ;
#111835=ORIENTED_EDGE ( 'NONE', *, *, #106173, .F. ) ;
#111836=DIRECTION ( 'NONE',  ( 0.000000000000000000, 1.000000000000000000, 0.000000000000000000 ) ) ;
#111837=EDGE_CURVE ( 'NONE', #54722, #36055, #64040, .T. ) ;
#111838=CONICAL_SURFACE ( 'NONE', #76241, 0.09999999999999999167, 0.003490658503988666988 ) ;
#111840=EDGE_CURVE ( 'NONE', #6241, #111738, #112164, .T. ) ;
#111841=PLANE ( 'NONE',  #9627 ) ;
#111843=ORIENTED_EDGE ( 'NONE', *, *, #29474, .F. ) ;
#111844=AXIS2_PLACEMENT_3D ( 'NONE', #112743, #121908, #74104 ) ;
#111845=CARTESIAN_POINT ( 'NONE',  ( 0.4499999999999569344, 2.500000000000000000, -2.065063509461102065 ) ) ;
#111846=CARTESIAN_POINT ( 'NONE',  ( -2.900000000000029221, 2.500000000000000000, -0.1000000000000022815 ) ) ;
#111847=ORIENTED_EDGE ( 'NONE', *, *, #67135, .F. ) ;
#111848=AXIS2_PLACEMENT_3D ( 'NONE', #82349, #84250, #74447 ) ;
#111849=AXIS2_PLACEMENT_3D ( 'NONE', #65384, #14342, #36604 ) ;
#111850=CIRCLE ( 'NONE', #97174, 0.09999999999999982514 ) ;
#111851=ORIENTED_EDGE ( 'NONE', *, *, #99977, .T. ) ;
#111852=ORIENTED_EDGE ( 'NONE', *, *, #74519, .T. ) ;
#111853=VERTEX_POINT ( 'NONE', #102699 ) ;
#111854=PLANE ( 'NONE',  #115765 ) ;
#111855=VECTOR ( 'NONE', #8305, 1000.000000000000000 ) ;
#111856=CARTESIAN_POINT ( 'NONE',  ( -8.750000000000010658, 2.500000000000000000, -1.472243186433550122 ) ) ;
#111857=CARTESIAN_POINT ( 'NONE',  ( 7.099999999999928590, 12.50000000000000000, -5.088040615133791356 ) ) ;
#111858=VECTOR ( 'NONE', #128172, 1000.000000000000000 ) ;
#111859=ORIENTED_EDGE ( 'NONE', *, *, #11788, .T. ) ;
#111860=CARTESIAN_POINT ( 'NONE',  ( -10.60000000000000142, 12.50000000000000000, 0.3464101615137736845 ) ) ;
#111861=AXIS2_PLACEMENT_3D ( 'NONE', #121463, #71739, #54498 ) ;
#111862=EDGE_LOOP ( 'NONE', ( #81927, #105780 ) ) ;
#111863=FACE_OUTER_BOUND ( 'NONE', #113619, .T. ) ;
#111864=CARTESIAN_POINT ( 'NONE',  ( -12.29999999999999716, 12.50000000000000000, 0.3464101615137776813 ) ) ;
#111865=DIRECTION ( 'NONE',  ( -0.000000000000000000, 1.000000000000000000, -0.000000000000000000 ) ) ;
#111866=FACE_OUTER_BOUND ( 'NONE', #51982, .T. ) ;
#111867=ORIENTED_EDGE ( 'NONE', *, *, #28964, .F. ) ;
#111868=EDGE_LOOP ( 'NONE', ( #103341, #87687, #90345, #68648 ) ) ;
#111869=ORIENTED_EDGE ( 'NONE', *, *, #74116, .F. ) ;
#111870=DIRECTION ( 'NONE',  ( 0.000000000000000000, 0.000000000000000000, 1.000000000000000000 ) ) ;
#111871=CARTESIAN_POINT ( 'NONE',  ( 12.09999999999990550, 12.50000000000000000, -3.572213422710612374 ) ) ;
#111872=CARTESIAN_POINT ( 'NONE',  ( -4.999999999999990230, 2.500000000000000000, -4.430127018922202176 ) ) ;
#111873=FACE_BOUND ( 'NONE', #5539, .T. ) ;
#111874=CARTESIAN_POINT ( 'NONE',  ( 11.64999999999990443, 2.500000000000000000, 1.472243186433545459 ) ) ;
#111875=CONICAL_SURFACE ( 'NONE', #67942, 0.09999999999999982514, 0.003490658503988666988 ) ;
#111876=DIRECTION ( 'NONE',  ( 0.000000000000000000, -0.9999939076577903929, 0.003490651415223739937 ) ) ;
#111877=FACE_OUTER_BOUND ( 'NONE', #47147, .T. ) ;
#111878=EDGE_CURVE ( 'NONE', #46373, #28259, #116348, .T. ) ;
#111879=DIRECTION ( 'NONE',  ( 0.000000000000000000, 0.000000000000000000, 1.000000000000000000 ) ) ;
#111880=AXIS2_PLACEMENT_3D ( 'NONE', #115932, #103552, #63625 ) ;
#111881=CARTESIAN_POINT ( 'NONE',  ( -1.650000000000034772, 12.50000000000000000, 1.407149913249508000 ) ) ;
#111882=PLANE ( 'NONE',  #122171 ) ;
#111883=ORIENTED_EDGE ( 'NONE', *, *, #113560, .F. ) ;
#111884=AXIS2_PLACEMENT_3D ( 'NONE', #110300, #122066, #101776 ) ;
#111885=AXIS2_PLACEMENT_3D ( 'NONE', #35115, #114927, #45570 ) ;
#111886=DIRECTION ( 'NONE',  ( 0.000000000000000000, 0.000000000000000000, 1.000000000000000000 ) ) ;
#111887=CARTESIAN_POINT ( 'NONE',  ( -4.350000000000023626, 2.500000000000000000, 6.148780366869520897 ) ) ;
#111888=VERTEX_POINT ( 'NONE', #104005 ) ;
#111889=ORIENTED_EDGE ( 'NONE', *, *, #87244, .T. ) ;
#111890=EDGE_CURVE ( 'NONE', #87436, #39393, #103367, .T. ) ;
#111891=DIRECTION ( 'NONE',  ( 0.000000000000000000, 1.000000000000000000, 0.000000000000000000 ) ) ;
#111892=CARTESIAN_POINT ( 'NONE',  ( 11.89999999999990798, 12.50000000000000000, 4.676537180435972552 ) ) ;
#111893=ADVANCED_FACE ( 'NONE', ( #4482 ), #66172, .T. ) ;
#111894=FACE_BOUND ( 'NONE', #52612, .T. ) ;
#111895=CARTESIAN_POINT ( 'NONE',  ( 2.499999999999948930, 12.50000000000000000, -5.022947341949754119 ) ) ;
#111896=VECTOR ( 'NONE', #39446, 1000.000000000000000 ) ;
#111897=AXIS2_PLACEMENT_3D ( 'NONE', #115090, #54901, #76494 ) ;
#111898=EDGE_LOOP ( 'NONE', ( #82350, #68451, #106518, #94121 ) ) ;
#111899=DIRECTION ( 'NONE',  ( -0.000000000000000000, 1.000000000000000000, -0.000000000000000000 ) ) ;
#111900=ADVANCED_FACE ( 'NONE', ( #74541 ), #43224, .T. ) ;
#111901=DIRECTION ( 'NONE',  ( 0.000000000000000000, 0.000000000000000000, 1.000000000000000000 ) ) ;
#111902=EDGE_LOOP ( 'NONE', ( #113609, #112027 ) ) ;
#111903=LINE ( 'NONE', #71315, #107553 ) ;
#111905=AXIS2_PLACEMENT_3D ( 'NONE', #38324, #80827, #109638 ) ;
#111906=AXIS2_PLACEMENT_3D ( 'NONE', #68272, #108198, #66972 ) ;
#111907=ORIENTED_EDGE ( 'NONE', *, *, #12285, .F. ) ;
#111908=DIRECTION ( 'NONE',  ( 0.000000000000000000, -0.9999939076577903929, 0.003490651415223739937 ) ) ;
#111909=DIRECTION ( 'NONE',  ( 0.000000000000000000, 1.000000000000000000, 0.000000000000000000 ) ) ;
#111910=ORIENTED_EDGE ( 'NONE', *, *, #19449, .T. ) ;
#111911=DIRECTION ( 'NONE',  ( 0.000000000000000000, -0.9999939076577903929, 0.003490651415223739937 ) ) ;
#111912=DIRECTION ( 'NONE',  ( 0.000000000000000000, -0.9999939076577903929, 0.003490651415223739937 ) ) ;
#111913=AXIS2_PLACEMENT_3D ( 'NONE', #94699, #104520, #62684 ) ;
#111914=DIRECTION ( 'NONE',  ( -0.000000000000000000, 1.000000000000000000, -0.000000000000000000 ) ) ;
#111915=ORIENTED_EDGE ( 'NONE', *, *, #13553, .T. ) ;
#111916=ORIENTED_EDGE ( 'NONE', *, *, #91412, .F. ) ;
#111917=DIRECTION ( 'NONE',  ( 0.000000000000000000, -0.9999939076577903929, 0.003490651415223739937 ) ) ;
#111918=CONICAL_SURFACE ( 'NONE', #5289, 0.09999999999999982514, 0.003490658503988666988 ) ;
#111919=ORIENTED_EDGE ( 'NONE', *, *, #62715, .F. ) ;
#111920=DIRECTION ( 'NONE',  ( -0.000000000000000000, 1.000000000000000000, -0.000000000000000000 ) ) ;
#111921=CARTESIAN_POINT ( 'NONE',  ( -7.500000000000001776, 2.500000000000000000, 9.000000000000001776 ) ) ;
#111922=EDGE_CURVE ( 'NONE', #113276, #29766, #30609, .T. ) ;
#111923=AXIS2_PLACEMENT_3D ( 'NONE', #91299, #121401, #71025 ) ;
#111924=DIRECTION ( 'NONE',  ( 0.000000000000000000, 0.000000000000000000, -1.000000000000000000 ) ) ;
#111925=VERTEX_POINT ( 'NONE', #114457 ) ;
#111926=AXIS2_PLACEMENT_3D ( 'NONE', #102961, #121973, #12642 ) ;
#111927=FACE_OUTER_BOUND ( 'NONE', #102922, .T. ) ;
#111928=DIRECTION ( 'NONE',  ( -0.000000000000000000, 1.000000000000000000, -0.000000000000000000 ) ) ;
#111929=DIRECTION ( 'NONE',  ( 0.000000000000000000, 1.000000000000000000, 0.000000000000000000 ) ) ;
#111930=CARTESIAN_POINT ( 'NONE',  ( -11.84999999999999609, 2.500000000000000000, 2.611473670974873151 ) ) ;
#111931=DIRECTION ( 'NONE',  ( -0.000000000000000000, -1.000000000000000000, -0.000000000000000000 ) ) ;
#111932=EDGE_CURVE ( 'NONE', #29267, #2432, #18055, .T. ) ;
#111933=FACE_OUTER_BOUND ( 'NONE', #80749, .T. ) ;
#111934=EDGE_CURVE ( 'NONE', #64926, #55907, #110022, .T. ) ;
#111935=CONICAL_SURFACE ( 'NONE', #28309, 0.1000000000000000472, 0.003490658503988666988 ) ;
#111937=AXIS2_PLACEMENT_3D ( 'NONE', #119635, #29995, #69912 ) ;
#111938=ORIENTED_EDGE ( 'NONE', *, *, #79445, .F. ) ;
#111939=AXIS2_PLACEMENT_3D ( 'NONE', #114063, #64307, #25671 ) ;
#111940=PLANE ( 'NONE',  #45369 ) ;
#111942=LINE ( 'NONE', #32104, #57712 ) ;
#111943=EDGE_CURVE ( 'NONE', #112113, #64505, #64712, .T. ) ;
#111944=CIRCLE ( 'NONE', #26261, 0.1000000000000002554 ) ;
#111945=ORIENTED_EDGE ( 'NONE', *, *, #23690, .T. ) ;
#111946=ORIENTED_EDGE ( 'NONE', *, *, #25908, .T. ) ;
#111947=EDGE_CURVE ( 'NONE', #5078, #119339, #99641, .T. ) ;
#111948=EDGE_LOOP ( 'NONE', ( #90769, #42301, #117292, #83744 ) ) ;
#111949=EDGE_CURVE ( 'NONE', #96192, #94402, #59959, .T. ) ;
#111950=CARTESIAN_POINT ( 'NONE',  ( -3.150000000000030109, 2.500000000000000000, -2.511473670974877948 ) ) ;
#111951=ADVANCED_FACE ( 'NONE', ( #86928 ), #15605, .T. ) ;
#111952=AXIS2_PLACEMENT_3D ( 'NONE', #100533, #52097, #22645 ) ;
#111953=DIRECTION ( 'NONE',  ( 0.000000000000000000, 0.000000000000000000, 1.000000000000000000 ) ) ;
#111954=CONICAL_SURFACE ( 'NONE', #101486, 0.1000000000000002554, 0.003490658503988666988 ) ;
#111955=FACE_OUTER_BOUND ( 'NONE', #108285, .T. ) ;
#111957=EDGE_CURVE ( 'NONE', #15249, #13248, #126741, .T. ) ;
#111958=DIRECTION ( 'NONE',  ( -0.000000000000000000, 1.000000000000000000, -0.000000000000000000 ) ) ;
#111959=CARTESIAN_POINT ( 'NONE',  ( -0.8000000000000381251, 2.500000000000000000, 4.430127018922196847 ) ) ;
#111960=CARTESIAN_POINT ( 'NONE',  ( 21.25101261094843963, 0.2446824650187501560, 4.189229355218854423 ) ) ;
#111961=CIRCLE ( 'NONE', #103636, 0.1000000000000000472 ) ;
#111962=DIRECTION ( 'NONE',  ( 0.000000000000000000, 0.000000000000000000, 1.000000000000000000 ) ) ;
#111963=DIRECTION ( 'NONE',  ( -0.000000000000000000, -1.000000000000000000, -0.000000000000000000 ) ) ;
#111964=FACE_OUTER_BOUND ( 'NONE', #17200, .T. ) ;
#111965=EDGE_CURVE ( 'NONE', #112226, #70902, #67256, .T. ) ;
#111966=ORIENTED_EDGE ( 'NONE', *, *, #13066, .T. ) ;
#111967=DIRECTION ( 'NONE',  ( -0.000000000000000000, 1.000000000000000000, -0.000000000000000000 ) ) ;
#111968=VERTEX_POINT ( 'NONE', #126219 ) ;
#111969=EDGE_LOOP ( 'NONE', ( #18679, #75357, #109901, #51559 ) ) ;
#111970=CARTESIAN_POINT ( 'NONE',  ( -10.20000000000000639, 2.500000000000000000, -3.983716857408421852 ) ) ;
#111971=CARTESIAN_POINT ( 'NONE',  ( -7.950000000000012612, 12.50000000000000000, 2.165063509461097713 ) ) ;
#111972=AXIS2_PLACEMENT_3D ( 'NONE', #57662, #95646, #76652 ) ;
#111973=CARTESIAN_POINT ( 'NONE',  ( -3.350000000000028511, 2.500000000000000000, 2.957883832488649389 ) ) ;
#111974=DIRECTION ( 'NONE',  ( 0.000000000000000000, 1.000000000000000000, 0.000000000000000000 ) ) ;
#111976=CARTESIAN_POINT ( 'NONE',  ( 4.599999999999940137, 12.50000000000000000, -4.395220292106239768 ) ) ;
#111977=CARTESIAN_POINT ( 'NONE',  ( 0.8499999999999536815, 2.500000000000000000, 6.495190528383297135 ) ) ;
#111978=DIRECTION ( 'NONE',  ( 0.000000000000000000, 0.000000000000000000, 1.000000000000000000 ) ) ;
#111979=ORIENTED_EDGE ( 'NONE', *, *, #52839, .T. ) ;
#111980=AXIS2_PLACEMENT_3D ( 'NONE', #18370, #36749, #87748 ) ;
#111981=AXIS2_PLACEMENT_3D ( 'NONE', #91280, #2910, #3544 ) ;
#111982=AXIS2_PLACEMENT_3D ( 'NONE', #84830, #26567, #75022 ) ;
#111983=ORIENTED_EDGE ( 'NONE', *, *, #44435, .T. ) ;
#111984=ORIENTED_EDGE ( 'NONE', *, *, #152, .F. ) ;
#111985=AXIS2_PLACEMENT_3D ( 'NONE', #27039, #66938, #106864 ) ;
#111986=ORIENTED_EDGE ( 'NONE', *, *, #25487, .T. ) ;
#111987=ORIENTED_EDGE ( 'NONE', *, *, #68372, .T. ) ;
#111988=FACE_OUTER_BOUND ( 'NONE', #52541, .T. ) ;
#111989=CARTESIAN_POINT ( 'NONE',  ( -6.650000000000015454, 12.50000000000000000, 2.857883832488649301 ) ) ;
#111990=CIRCLE ( 'NONE', #91052, 0.1000000000000002554 ) ;
#111991=FACE_OUTER_BOUND ( 'NONE', #7437, .T. ) ;
#111992=ADVANCED_FACE ( 'NONE', ( #76484 ), #35279, .T. ) ;
#111993=DIRECTION ( 'NONE',  ( 0.000000000000000000, 0.000000000000000000, 1.000000000000000000 ) ) ;
#111994=AXIS2_PLACEMENT_3D ( 'NONE', #10323, #1144, #40449 ) ;
#111995=DIRECTION ( 'NONE',  ( 0.000000000000000000, -0.9999939076577903929, 0.003490651415223739937 ) ) ;
#111996=ORIENTED_EDGE ( 'NONE', *, *, #80313, .F. ) ;
#111997=CARTESIAN_POINT ( 'NONE',  ( 2.099999999999950351, 12.50000000000000000, 0.06509327318403515528 ) ) ;
#111998=DIRECTION ( 'NONE',  ( 0.000000000000000000, 1.000000000000000000, 0.000000000000000000 ) ) ;
#111999=DIRECTION ( 'NONE',  ( -0.000000000000000000, 1.000000000000000000, -0.000000000000000000 ) ) ;
#112000=DIRECTION ( 'NONE',  ( -4.274815082592931898E-19, -0.9999939076577903929, -0.003490651415223739937 ) ) ;
#112001=DIRECTION ( 'NONE',  ( 0.000000000000000000, 0.000000000000000000, 1.000000000000000000 ) ) ;
#112002=EDGE_CURVE ( 'NONE', #76525, #90431, #55711, .T. ) ;
#112003=VERTEX_POINT ( 'NONE', #36571 ) ;
#112004=AXIS2_PLACEMENT_3D ( 'NONE', #117320, #85319, #85946 ) ;
#112005=AXIS2_PLACEMENT_3D ( 'NONE', #50569, #112082, #110144 ) ;
#112006=EDGE_LOOP ( 'NONE', ( #110201, #19151, #8829, #92968 ) ) ;
#112007=EDGE_LOOP ( 'NONE', ( #79512, #65820, #90799, #13129 ) ) ;
#112008=DIRECTION ( 'NONE',  ( -0.000000000000000000, -1.000000000000000000, -0.000000000000000000 ) ) ;
#112009=EDGE_LOOP ( 'NONE', ( #99456, #110350, #75670, #82529 ) ) ;
#112010=CARTESIAN_POINT ( 'NONE',  ( -5.800000000000018474, 2.500000000000000000, 4.330127018922196314 ) ) ;
#112011=DIRECTION ( 'NONE',  ( 0.000000000000000000, 1.000000000000000000, 0.000000000000000000 ) ) ;
#112012=VERTEX_POINT ( 'NONE', #116383 ) ;
#112013=CARTESIAN_POINT ( 'NONE',  ( 15.39999999999989200, 2.500000000000000000, 0.7928203230275495672 ) ) ;
#112014=DIRECTION ( 'NONE',  ( 0.000000000000000000, 0.000000000000000000, -1.000000000000000000 ) ) ;
#112016=CARTESIAN_POINT ( 'NONE',  ( 9.399999999999915090, 2.500000000000000000, 4.083716857408421497 ) ) ;
#112017=CIRCLE ( 'NONE', #26247, 0.1000000000000000472 ) ;
#112018=CARTESIAN_POINT ( 'NONE',  ( 12.09999999999990550, 2.500000000000000000, 4.330127018922196314 ) ) ;
#112019=CIRCLE ( 'NONE', #15761, 0.06509327318403745899 ) ;
#112020=ORIENTED_EDGE ( 'NONE', *, *, #111024, .F. ) ;
#112021=ORIENTED_EDGE ( 'NONE', *, *, #70738, .F. ) ;
#112022=CARTESIAN_POINT ( 'NONE',  ( 15.39999999999989200, 12.50000000000000000, 0.6928203230275494784 ) ) ;
#112023=CARTESIAN_POINT ( 'NONE',  ( 4.149999999999939959, 2.500000000000000000, 1.572243186433545548 ) ) ;
#112024=CARTESIAN_POINT ( 'NONE',  ( -10.85000000000000142, 12.50000000000000000, -7.188010851410850499 ) ) ;
#112025=CARTESIAN_POINT ( 'NONE',  ( -1.850000000000033840, 12.50000000000000000, 1.753560074763284016 ) ) ;
#112026=EDGE_CURVE ( 'NONE', #40133, #4247, #47320, .T. ) ;
#112027=ORIENTED_EDGE ( 'NONE', *, *, #18385, .T. ) ;
#112028=CIRCLE ( 'NONE', #74371, 0.06509327318403745899 ) ;
#112029=EDGE_LOOP ( 'NONE', ( #86562, #24768 ) ) ;
#112030=CARTESIAN_POINT ( 'NONE',  ( -10.85000000000000142, 2.500000000000000000, -1.472243186433546125 ) ) ;
#112031=DIRECTION ( 'NONE',  ( 0.000000000000000000, 0.000000000000000000, 1.000000000000000000 ) ) ;
#112032=FACE_OUTER_BOUND ( 'NONE', #53383, .T. ) ;
#112033=PLANE ( 'NONE',  #61450 ) ;
#112034=EDGE_LOOP ( 'NONE', ( #53484, #69555, #92841, #21607 ) ) ;
#112035=CONICAL_SURFACE ( 'NONE', #55597, 0.09999999999999982514, 0.003490658503988666988 ) ;
#112036=ADVANCED_FACE ( 'NONE', ( #37207 ), #5533, .T. ) ;
#112037=DIRECTION ( 'NONE',  ( 0.000000000000000000, 0.000000000000000000, -1.000000000000000000 ) ) ;
#112038=CONICAL_SURFACE ( 'NONE', #32649, 0.1000000000000000472, 0.003490658503988666988 ) ;
#112039=DIRECTION ( 'NONE',  ( 0.000000000000000000, 0.000000000000000000, 1.000000000000000000 ) ) ;
#112040=CIRCLE ( 'NONE', #116042, 0.09999999999999982514 ) ;
#112041=ORIENTED_EDGE ( 'NONE', *, *, #77361, .F. ) ;
#112042=EDGE_CURVE ( 'NONE', #42690, #62384, #66005, .T. ) ;
#112043=CARTESIAN_POINT ( 'NONE',  ( 12.29999999999990123, 2.500000000000000000, 0.3464101615137735735 ) ) ;
#112045=EDGE_LOOP ( 'NONE', ( #94705, #122406, #94873, #49504 ) ) ;
#112046=CARTESIAN_POINT ( 'NONE',  ( 9.149999999999918643, 12.50000000000000000, -6.430097255199264339 ) ) ;
#112047=ORIENTED_EDGE ( 'NONE', *, *, #78371, .F. ) ;
#112049=CARTESIAN_POINT ( 'NONE',  ( 10.84999999999990905, 2.500000000000000000, 2.857883832488649301 ) ) ;
#112050=EDGE_CURVE ( 'NONE', #104598, #63506, #118412, .T. ) ;
#112051=ORIENTED_EDGE ( 'NONE', *, *, #46314, .T. ) ;
#112052=ORIENTED_EDGE ( 'NONE', *, *, #80567, .T. ) ;
#112053=EDGE_CURVE ( 'NONE', #93285, #79041, #24327, .T. ) ;
#112054=CARTESIAN_POINT ( 'NONE',  ( 14.34999999999989306, 2.500000000000000000, -1.918653347947326004 ) ) ;
#112055=CARTESIAN_POINT ( 'NONE',  ( 13.09999999999989839, 2.500000000000000000, -0.4464101615137783252 ) ) ;
#112056=CIRCLE ( 'NONE', #91121, 0.09999999999999982514 ) ;
#112057=CARTESIAN_POINT ( 'NONE',  ( -14.14999999999998792, 12.50000000000000000, -1.407149913249510442 ) ) ;
#112059=CARTESIAN_POINT ( 'NONE',  ( -6.650000000000018119, 12.50000000000000000, -7.188010851410854052 ) ) ;
#112060=PLANE ( 'NONE',  #15901 ) ;
#112061=CARTESIAN_POINT ( 'NONE',  ( -7.050000000000013145, 12.50000000000000000, 2.165063509461097713 ) ) ;
#112062=LINE ( 'NONE', #22408, #51527 ) ;
#112063=DIRECTION ( 'NONE',  ( 0.000000000000000000, -0.000000000000000000, 1.000000000000000000 ) ) ;
#112064=CONICAL_SURFACE ( 'NONE', #72365, 0.1000000000000000472, 0.003490658503988666988 ) ;
#112065=VECTOR ( 'NONE', #18674, 1000.000000000000000 ) ;
#112066=ORIENTED_EDGE ( 'NONE', *, *, #100229, .F. ) ;
#112067=ORIENTED_EDGE ( 'NONE', *, *, #129238, .T. ) ;
#112068=CARTESIAN_POINT ( 'NONE',  ( 6.049999999999932321, 2.500000000000000000, 6.841600689897072485 ) ) ;
#112069=ORIENTED_EDGE ( 'NONE', *, *, #27275, .F. ) ;
#112070=CARTESIAN_POINT ( 'NONE',  ( 9.199999999999915801, 2.500000000000000000, 4.230127018922196669 ) ) ;
#112071=CARTESIAN_POINT ( 'NONE',  ( -10.20000000000000462, 12.50000000000000000, 0.3464101615137735735 ) ) ;
#112072=FACE_OUTER_BOUND ( 'NONE', #109106, .T. ) ;
#112073=ORIENTED_EDGE ( 'NONE', *, *, #58101, .F. ) ;
#112074=ORIENTED_EDGE ( 'NONE', *, *, #29784, .T. ) ;
#112075=FACE_BOUND ( 'NONE', #85933, .T. ) ;
#112076=ORIENTED_EDGE ( 'NONE', *, *, #89472, .F. ) ;
#112077=CARTESIAN_POINT ( 'NONE',  ( -11.84999999999999609, 2.500000000000000000, 1.818653347947321475 ) ) ;
#112078=CARTESIAN_POINT ( 'NONE',  ( -6.250000000000019540, 12.50000000000000000, -7.253104124594891289 ) ) ;
#112079=AXIS2_PLACEMENT_3D ( 'NONE', #5124, #5753, #115066 ) ;
#112080=CARTESIAN_POINT ( 'NONE',  ( -5.850000000000021849, 2.500000000000000000, -7.088010851410853519 ) ) ;
#112081=LINE ( 'NONE', #102264, #59784 ) ;
#112082=DIRECTION ( 'NONE',  ( 0.000000000000000000, 1.000000000000000000, 0.000000000000000000 ) ) ;
#112083=VECTOR ( 'NONE', #36618, 1000.000000000000000 ) ;
#112084=AXIS2_PLACEMENT_3D ( 'NONE', #97894, #76976, #48163 ) ;
#112085=DIRECTION ( 'NONE',  ( 0.000000000000000000, 0.000000000000000000, 1.000000000000000000 ) ) ;
#112086=LINE ( 'NONE', #72807, #30983 ) ;
#112087=DIRECTION ( 'NONE',  ( -4.274815082592931898E-19, -0.9999939076577903929, -0.003490651415223739937 ) ) ;
#112088=DIRECTION ( 'NONE',  ( -0.000000000000000000, -1.000000000000000000, -0.000000000000000000 ) ) ;
#112089=CARTESIAN_POINT ( 'NONE',  ( 11.84999999999990372, 2.500000000000000000, 1.718653347947321386 ) ) ;
#112090=DIRECTION ( 'NONE',  ( 0.000000000000000000, -0.9999939076577903929, 0.003490651415223739937 ) ) ;
#112091=ADVANCED_FACE ( 'NONE', ( #105935 ), #95437, .T. ) ;
#112092=ORIENTED_EDGE ( 'NONE', *, *, #19555, .T. ) ;
#112093=VERTEX_POINT ( 'NONE', #6407 ) ;
#112094=ORIENTED_EDGE ( 'NONE', *, *, #118135, .T. ) ;
#112096=EDGE_LOOP ( 'NONE', ( #123491, #62399 ) ) ;
#112097=DIRECTION ( 'NONE',  ( 0.000000000000000000, 1.000000000000000000, 0.000000000000000000 ) ) ;
#112098=ADVANCED_FACE ( 'NONE', ( #47297 ), #106832, .T. ) ;
#112099=CARTESIAN_POINT ( 'NONE',  ( 6.899999999999928413, 2.500000000000000000, -4.083716857408426826 ) ) ;
#112100=ADVANCED_FACE ( 'NONE', ( #107499 ), #57787, .T. ) ;
#112101=ORIENTED_EDGE ( 'NONE', *, *, #42393, .T. ) ;
#112102=VERTEX_POINT ( 'NONE', #56450 ) ;
#112103=ORIENTED_EDGE ( 'NONE', *, *, #39930, .T. ) ;
#112104=ADVANCED_FACE ( 'NONE', ( #7345 ), #34814, .T. ) ;
#112106=EDGE_CURVE ( 'NONE', #79005, #10181, #106212, .T. ) ;
#112107=DIRECTION ( 'NONE',  ( 0.000000000000000000, 1.000000000000000000, 0.000000000000000000 ) ) ;
#112108=CARTESIAN_POINT ( 'NONE',  ( 2.899999999999944844, 2.500000000000000000, 4.922947341949748257 ) ) ;
#112109=EDGE_CURVE ( 'NONE', #49224, #18575, #51529, .T. ) ;
#112110=CARTESIAN_POINT ( 'NONE',  ( 32.27737261621599885, -1.406459146828822782, -4.686451385768223510 ) ) ;
#112112=DIRECTION ( 'NONE',  ( 0.000000000000000000, 1.000000000000000000, 0.000000000000000000 ) ) ;
#112113=VERTEX_POINT ( 'NONE', #57764 ) ;
#112114=CARTESIAN_POINT ( 'NONE',  ( 6.449999999999931788, 2.500000000000000000, -6.248780366869526759 ) ) ;
#112115=EDGE_CURVE ( 'NONE', #116826, #21551, #68233, .T. ) ;
#112116=VERTEX_POINT ( 'NONE', #27624 ) ;
#112118=AXIS2_PLACEMENT_3D ( 'NONE', #32900, #112738, #100970 ) ;
#112119=EDGE_LOOP ( 'NONE', ( #127808, #127786, #88088, #74271 ) ) ;
#112120=VERTEX_POINT ( 'NONE', #67550 ) ;
#112121=CARTESIAN_POINT ( 'NONE',  ( -11.44999999999999751, 2.500000000000000000, 6.941600689897073018 ) ) ;
#112122=( BOUNDED_SURFACE ( )  B_SPLINE_SURFACE ( 3, 2, ( 
 ( #8333, #67902, #117622 ),
 ( #27983, #28639, #18153 ),
 ( #111539, #58099, #2212 ),
 ( #109100, #39763, #89482 ),
 ( #9631, #98004, #12675 ),
 ( #38469, #112186, #119571 ),
 ( #98637, #79656, #118939 ),
 ( #8974, #48267, #42158 ),
 ( #71608, #122012, #118295 ),
 ( #82074, #88163, #52611 ),
 ( #21889, #61809, #88833 ),
 ( #48928, #29283, #101728 ),
 ( #49572, #12040, #62457 ),
 ( #128125, #128791, #72275 ) ),
 .UNSPECIFIED., .F., .F., .F. ) 
 B_SPLINE_SURFACE_WITH_KNOTS ( ( 4, 2, 2, 2, 2, 2, 4 ),
 ( 3, 3 ),
 ( 0.000000000000000000, 0.001744612550434158091, 0.002616918825651237245, 0.003489225100868316182, 0.005233837651302474490, 0.006106143926519553428, 0.006978450201736632365 ),
 ( 0.000000000000000000, 1.000000000000000000 ),
 .UNSPECIFIED. ) 
 GEOMETRIC_REPRESENTATION_ITEM ( )  RATIONAL_B_SPLINE_SURFACE ( (
 ( 1.000000000000000000, 0.7318752858502195480, 1.000000000000000000),
 ( 1.000000000000000000, 0.7270130115578816721, 1.000000000000000000),
 ( 1.000000000000000000, 0.7223762446139350146, 1.000000000000000000),
 ( 1.000000000000000000, 0.7156127915551184770, 1.000000000000000000),
 ( 1.000000000000000000, 0.7133893117691979535, 1.000000000000000000),
 ( 1.000000000000000000, 0.7090389252573886525, 1.000000000000000000),
 ( 1.000000000000000000, 0.7069297463491840405, 1.000000000000000000),
 ( 1.000000000000000000, 0.7010696893200119018, 1.000000000000000000),
 ( 1.000000000000000000, 0.6977361265598627238, 1.000000000000000000),
 ( 1.000000000000000000, 0.6948030504688554876, 1.000000000000000000),
 ( 1.000000000000000000, 0.6942033558615359201, 1.000000000000000000),
 ( 1.000000000000000000, 0.6937817651808704245, 1.000000000000000000),
 ( 1.000000000000000000, 0.6939284133496994578, 1.000000000000000000),
 ( 1.000000000000000000, 0.6944177883068215484, 1.000000000000000000) ) ) 
 REPRESENTATION_ITEM ( '' )  SURFACE ( )  );
#112123=VERTEX_POINT ( 'NONE', #7995 ) ;
#112124=EDGE_LOOP ( 'NONE', ( #117338, #67662 ) ) ;
#112125=ORIENTED_EDGE ( 'NONE', *, *, #89059, .F. ) ;
#112126=CARTESIAN_POINT ( 'NONE',  ( 5.399999999999935518, 2.500000000000000000, -4.330127018922201643 ) ) ;
#112127=CONICAL_SURFACE ( 'NONE', #128869, 0.09999999999999982514, 0.003490658503988666988 ) ;
#112128=CIRCLE ( 'NONE', #32721, 0.06509327318403745899 ) ;
#112129=DIRECTION ( 'NONE',  ( -0.000000000000000000, 1.000000000000000000, -0.000000000000000000 ) ) ;
#112130=DIRECTION ( 'NONE',  ( 0.000000000000000000, 1.000000000000000000, 0.000000000000000000 ) ) ;
#112131=CARTESIAN_POINT ( 'NONE',  ( 11.44999999999991047, 2.500000000000000000, -2.411473670974877859 ) ) ;
#112132=LINE ( 'NONE', #110821, #17732 ) ;
#112133=DIRECTION ( 'NONE',  ( 0.000000000000000000, 0.000000000000000000, 1.000000000000000000 ) ) ;
#112134=CARTESIAN_POINT ( 'NONE',  ( -8.300000000000011369, 12.50000000000000000, 0.06509327318403515528 ) ) ;
#112136=ORIENTED_EDGE ( 'NONE', *, *, #97152, .T. ) ;
#112137=CARTESIAN_POINT ( 'NONE',  ( -2.100000000000033396, 12.50000000000000000, -4.957854068765716882 ) ) ;
#112138=CONICAL_SURFACE ( 'NONE', #3465, 0.09999999999999982514, 0.003490658503988666988 ) ;
#112139=ORIENTED_EDGE ( 'NONE', *, *, #1527, .T. ) ;
#112140=FACE_OUTER_BOUND ( 'NONE', #127537, .T. ) ;
#112141=VERTEX_POINT ( 'NONE', #98966 ) ;
#112142=LINE ( 'NONE', #891, #73976 ) ;
#112143=ORIENTED_EDGE ( 'NONE', *, *, #61643, .T. ) ;
#112145=CARTESIAN_POINT ( 'NONE',  ( -9.150000000000009237, 2.500000000000000000, 2.165063509461097713 ) ) ;
#112146=VERTEX_POINT ( 'NONE', #8626 ) ;
#112147=ORIENTED_EDGE ( 'NONE', *, *, #75856, .T. ) ;
#112148=FACE_OUTER_BOUND ( 'NONE', #68696, .T. ) ;
#112149=FACE_OUTER_BOUND ( 'NONE', #116357, .T. ) ;
#112150=CARTESIAN_POINT ( 'NONE',  ( 6.899999999999928413, 12.50000000000000000, -4.676537180435977881 ) ) ;
#112151=AXIS2_PLACEMENT_3D ( 'NONE', #9691, #110464, #49636 ) ;
#112152=DIRECTION ( 'NONE',  ( -0.000000000000000000, -1.000000000000000000, -0.000000000000000000 ) ) ;
#112153=CARTESIAN_POINT ( 'NONE',  ( -4.350000000000023626, 12.50000000000000000, -1.753560074763288457 ) ) ;
#112154=EDGE_CURVE ( 'NONE', #103978, #74727, #43311, .T. ) ;
#112155=VERTEX_POINT ( 'NONE', #108772 ) ;
#112156=CONICAL_SURFACE ( 'NONE', #49474, 0.1000000000000000056, 0.003490658503988666988 ) ;
#112157=CARTESIAN_POINT ( 'NONE',  ( 2.500000000000002220, -2.500000000000000000, 9.000000000000001776 ) ) ;
#112158=AXIS2_PLACEMENT_3D ( 'NONE', #7099, #116410, #126897 ) ;
#112159=AXIS2_PLACEMENT_3D ( 'NONE', #11912, #13839, #33509 ) ;
#112161=AXIS2_PLACEMENT_3D ( 'NONE', #77439, #18517, #17193 ) ;
#112162=DIRECTION ( 'NONE',  ( -4.274815082592931898E-19, -0.9999939076577903929, -0.003490651415223739937 ) ) ;
#112163=FACE_OUTER_BOUND ( 'NONE', #52801, .T. ) ;
#112164=CIRCLE ( 'NONE', #72452, 0.1000000000000002554 ) ;
#112165=LINE ( 'NONE', #29733, #103997 ) ;
#112166=CARTESIAN_POINT ( 'NONE',  ( -15.39999999999998082, 12.50000000000000000, 0.6928203230275518099 ) ) ;
#112167=DIRECTION ( 'NONE',  ( -0.000000000000000000, 1.000000000000000000, -0.000000000000000000 ) ) ;
#112168=LINE ( 'NONE', #103640, #62815 ) ;
#112169=CARTESIAN_POINT ( 'NONE',  ( -10.85000000000000142, 12.50000000000000000, -2.857883832488649745 ) ) ;
#112170=EDGE_LOOP ( 'NONE', ( #16639, #16506 ) ) ;
#112171=AXIS2_PLACEMENT_3D ( 'NONE', #76785, #97699, #87866 ) ;
#112172=DIRECTION ( 'NONE',  ( 0.000000000000000000, 0.000000000000000000, 1.000000000000000000 ) ) ;
#112173=AXIS2_PLACEMENT_3D ( 'NONE', #60127, #28721, #99393 ) ;
#112174=AXIS2_PLACEMENT_3D ( 'NONE', #85188, #125120, #95657 ) ;
#112175=LINE ( 'NONE', #32984, #109134 ) ;
#112176=DIRECTION ( 'NONE',  ( 0.000000000000000000, -0.9999939076577903929, 0.003490651415223739937 ) ) ;
#112177=EDGE_LOOP ( 'NONE', ( #103918, #23712 ) ) ;
#112178=ORIENTED_EDGE ( 'NONE', *, *, #36425, .F. ) ;
#112179=CARTESIAN_POINT ( 'NONE',  ( -7.950000000000012612, 2.500000000000000000, 2.065063509461097624 ) ) ;
#112180=ORIENTED_EDGE ( 'NONE', *, *, #108255, .F. ) ;
#112181=ORIENTED_EDGE ( 'NONE', *, *, #78727, .F. ) ;
#112182=LINE ( 'NONE', #74191, #82331 ) ;
#112183=VERTEX_POINT ( 'NONE', #87840 ) ;
#112184=DIRECTION ( 'NONE',  ( 0.000000000000000000, 0.000000000000000000, -1.000000000000000000 ) ) ;
#112185=DIRECTION ( 'NONE',  ( 0.000000000000000000, -0.9999939076577903929, 0.003490651415223739937 ) ) ;
#112186=CARTESIAN_POINT ( 'NONE',  ( 18.98912670146768633, 2.543039972612955335, 4.488908218018861973 ) ) ;
#112187=EDGE_LOOP ( 'NONE', ( #89584, #120688, #127052, #11920 ) ) ;
#112188=EDGE_CURVE ( 'NONE', #40568, #124666, #129000, .T. ) ;
#112189=DIRECTION ( 'NONE',  ( 0.000000000000000000, 0.000000000000000000, 1.000000000000000000 ) ) ;
#112190=LINE ( 'NONE', #93204, #91311 ) ;
#112191=ADVANCED_FACE ( 'NONE', ( #96366 ), #91319, .T. ) ;
#112192=ADVANCED_FACE ( 'NONE', ( #58414 ), #78821, .T. ) ;
#112193=VERTEX_POINT ( 'NONE', #68205 ) ;
#112194=VECTOR ( 'NONE', #58967, 1000.000000000000000 ) ;
#112195=ORIENTED_EDGE ( 'NONE', *, *, #28854, .T. ) ;
#112196=AXIS2_PLACEMENT_3D ( 'NONE', #24896, #115848, #113929 ) ;
#112197=EDGE_LOOP ( 'NONE', ( #127533, #27554, #35795, #69184 ) ) ;
#112198=CARTESIAN_POINT ( 'NONE',  ( -0.6500000000000398792, 2.500000000000000000, -6.841600689897078702 ) ) ;
#112199=LINE ( 'NONE', #52625, #106397 ) ;
#112200=EDGE_CURVE ( 'NONE', #90179, #39201, #110099, .T. ) ;
#112201=EDGE_CURVE ( 'NONE', #46879, #71600, #46644, .T. ) ;
#112202=DIRECTION ( 'NONE',  ( 0.000000000000000000, 0.000000000000000000, 1.000000000000000000 ) ) ;
#112203=EDGE_CURVE ( 'NONE', #6770, #89861, #126827, .T. ) ;
#112204=FACE_BOUND ( 'NONE', #43249, .T. ) ;
#112205=ORIENTED_EDGE ( 'NONE', *, *, #117075, .T. ) ;
#112206=EDGE_CURVE ( 'NONE', #84673, #20142, #88491, .T. ) ;
#112207=FACE_OUTER_BOUND ( 'NONE', #24878, .T. ) ;
#112209=VERTEX_POINT ( 'NONE', #9296 ) ;
#112210=CIRCLE ( 'NONE', #78778, 0.1000000000000002554 ) ;
#112211=CIRCLE ( 'NONE', #124721, 0.09999999999999982514 ) ;
#112212=DIRECTION ( 'NONE',  ( 0.000000000000000000, 0.000000000000000000, 1.000000000000000000 ) ) ;
#112213=FACE_OUTER_BOUND ( 'NONE', #46962, .T. ) ;
#112214=CARTESIAN_POINT ( 'NONE',  ( 10.84999999999990905, 12.50000000000000000, -7.122917578226816815 ) ) ;
#112215=DIRECTION ( 'NONE',  ( 0.000000000000000000, 0.000000000000000000, -1.000000000000000000 ) ) ;
#112216=FACE_OUTER_BOUND ( 'NONE', #119396, .T. ) ;
#112217=CIRCLE ( 'NONE', #122673, 0.09999999999999982514 ) ;
#112218=ADVANCED_FACE ( 'NONE', ( #49241 ), #3584, .T. ) ;
#112219=CARTESIAN_POINT ( 'NONE',  ( -10.65000000000000391, 2.500000000000000000, -1.718653347947322052 ) ) ;
#112220=FACE_OUTER_BOUND ( 'NONE', #90191, .T. ) ;
#112221=AXIS2_PLACEMENT_3D ( 'NONE', #19754, #99602, #59697 ) ;
#112222=AXIS2_PLACEMENT_3D ( 'NONE', #2546, #31402, #52317 ) ;
#112223=ORIENTED_EDGE ( 'NONE', *, *, #114426, .F. ) ;
#112224=VERTEX_POINT ( 'NONE', #62275 ) ;
#112225=VERTEX_POINT ( 'NONE', #121818 ) ;
#112226=VERTEX_POINT ( 'NONE', #40051 ) ;
#112227=DIRECTION ( 'NONE',  ( 0.000000000000000000, 0.000000000000000000, -1.000000000000000000 ) ) ;
#112228=DIRECTION ( 'NONE',  ( -4.274815082592931898E-19, -0.9999939076577903929, -0.003490651415223739937 ) ) ;
#112229=CARTESIAN_POINT ( 'NONE',  ( -15.19999999999998330, 2.500000000000000000, 0.2464101615137758439 ) ) ;
#112230=ORIENTED_EDGE ( 'NONE', *, *, #66010, .T. ) ;
#112231=FACE_BOUND ( 'NONE', #78627, .T. ) ;
#112232=CARTESIAN_POINT ( 'NONE',  ( 0.8499999999999545697, 2.500000000000000000, 2.857883832488649301 ) ) ;
#112233=FACE_OUTER_BOUND ( 'NONE', #28108, .T. ) ;
#112234=CARTESIAN_POINT ( 'NONE',  ( -3.749999999999991118, 2.500000000000000000, 2.065063509461097624 ) ) ;
#112235=CARTESIAN_POINT ( 'NONE',  ( 13.54999999999990123, 2.500000000000000000, 1.718653347947321386 ) ) ;
#112236=CARTESIAN_POINT ( 'NONE',  ( -12.49999999999995914, 12.50000000000000000, 1.843143693225357538E-15 ) ) ;
#112237=CARTESIAN_POINT ( 'NONE',  ( -7.050000000000013145, 2.500000000000000000, 2.065063509461097624 ) ) ;
#112238=FACE_OUTER_BOUND ( 'NONE', #124432, .T. ) ;
#112239=CARTESIAN_POINT ( 'NONE',  ( -2.900000000000030109, 2.500000000000000000, -3.637306695894650055 ) ) ;
#112240=EDGE_CURVE ( 'NONE', #117617, #30567, #39118, .T. ) ;
#112241=CARTESIAN_POINT ( 'NONE',  ( -5.450000000000023270, 12.50000000000000000, -2.165063509461101710 ) ) ;
#112242=CIRCLE ( 'NONE', #34896, 0.06509327318403745899 ) ;
#112243=CIRCLE ( 'NONE', #74871, 0.1000000000000002554 ) ;
#112244=CIRCLE ( 'NONE', #101782, 0.06509327318403745899 ) ;
#112245=VERTEX_POINT ( 'NONE', #69491 ) ;
#112247=CIRCLE ( 'NONE', #41247, 0.06509327318403745899 ) ;
#112248=ORIENTED_EDGE ( 'NONE', *, *, #101408, .T. ) ;
#112249=ORIENTED_EDGE ( 'NONE', *, *, #48374, .T. ) ;
#112250=VERTEX_POINT ( 'NONE', #70790 ) ;
#112251=ORIENTED_EDGE ( 'NONE', *, *, #112106, .T. ) ;
#112252=FACE_OUTER_BOUND ( 'NONE', #38240, .T. ) ;
#112253=EDGE_CURVE ( 'NONE', #23452, #1757, #24421, .T. ) ;
#112254=ORIENTED_EDGE ( 'NONE', *, *, #20772, .F. ) ;
#112255=CIRCLE ( 'NONE', #30700, 0.06509327318403745899 ) ;
#112256=VERTEX_POINT ( 'NONE', #79343 ) ;
#112257=EDGE_CURVE ( 'NONE', #68589, #63643, #101795, .T. ) ;
#112258=AXIS2_PLACEMENT_3D ( 'NONE', #108515, #59447, #30625 ) ;
#112259=AXIS2_PLACEMENT_3D ( 'NONE', #11860, #9939, #101546 ) ;
#112260=EDGE_CURVE ( 'NONE', #48344, #129288, #97569, .T. ) ;
#112261=CARTESIAN_POINT ( 'NONE',  ( -10.20000000000000462, 2.500000000000000000, 4.676537180435972552 ) ) ;
#112262=CARTESIAN_POINT ( 'NONE',  ( 7.499999999999925393, 12.50000000000000000, 5.022947341949748790 ) ) ;
#112263=DIRECTION ( 'NONE',  ( -0.000000000000000000, 1.000000000000000000, -0.000000000000000000 ) ) ;
#112264=DIRECTION ( 'NONE',  ( 0.000000000000000000, -0.9999939076577903929, 0.003490651415223739937 ) ) ;
#112265=CIRCLE ( 'NONE', #26580, 0.1000000000000000472 ) ;
#112267=ORIENTED_EDGE ( 'NONE', *, *, #87831, .T. ) ;
#112268=CARTESIAN_POINT ( 'NONE',  ( 4.199999999999938005, 2.500000000000000000, 4.230127018922196669 ) ) ;
#112269=CIRCLE ( 'NONE', #85063, 0.06509327318403745899 ) ;
#112270=EDGE_CURVE ( 'NONE', #71534, #34595, #87100, .T. ) ;
#112271=EDGE_CURVE ( 'NONE', #47988, #1124, #16076, .T. ) ;
#112272=ORIENTED_EDGE ( 'NONE', *, *, #109830, .F. ) ;
#112273=CIRCLE ( 'NONE', #5630, 0.09999999999999999167 ) ;
#112274=VECTOR ( 'NONE', #54426, 1000.000000000000000 ) ;
#112275=EDGE_CURVE ( 'NONE', #74808, #6403, #95533, .T. ) ;
#112276=ORIENTED_EDGE ( 'NONE', *, *, #65210, .F. ) ;
#112277=CARTESIAN_POINT ( 'NONE',  ( 8.149999999999920419, 12.50000000000000000, -1.818653347947325916 ) ) ;
#112278=CARTESIAN_POINT ( 'NONE',  ( 6.649999999999927525, 12.50000000000000000, 2.099970236277060032 ) ) ;
#112279=ORIENTED_EDGE ( 'NONE', *, *, #73455, .T. ) ;
#112280=EDGE_CURVE ( 'NONE', #56703, #123357, #116440, .T. ) ;
#112281=EDGE_LOOP ( 'NONE', ( #17902, #123714, #18001, #49206 ) ) ;
#112282=CARTESIAN_POINT ( 'NONE',  ( -4.350000000000023626, 2.500000000000000000, -1.718653347947325827 ) ) ;
#112283=DIRECTION ( 'NONE',  ( 0.000000000000000000, 0.000000000000000000, 1.000000000000000000 ) ) ;
#112284=CARTESIAN_POINT ( 'NONE',  ( -5.450000000000019718, 2.500000000000000000, 2.065063509461097624 ) ) ;
#112285=CARTESIAN_POINT ( 'NONE',  ( -13.14999999999999147, 12.50000000000000000, -1.883746621131361376 ) ) ;
#112286=DIRECTION ( 'NONE',  ( 0.000000000000000000, 0.000000000000000000, 1.000000000000000000 ) ) ;
#112287=CONICAL_SURFACE ( 'NONE', #20246, 0.1000000000000000056, 0.003490658503988666988 ) ;
#112288=ORIENTED_EDGE ( 'NONE', *, *, #14063, .F. ) ;
#112289=PLANE ( 'NONE',  #32364 ) ;
#112291=CARTESIAN_POINT ( 'NONE',  ( 14.79999999999989235, 2.500000000000000000, 0.2464101615137735679 ) ) ;
#112292=LINE ( 'NONE', #122113, #18043 ) ;
#112294=DIRECTION ( 'NONE',  ( 0.000000000000000000, 0.000000000000000000, 1.000000000000000000 ) ) ;
#112295=CARTESIAN_POINT ( 'NONE',  ( 9.149999999999916866, 12.50000000000000000, -1.407149913249512663 ) ) ;
#112296=ORIENTED_EDGE ( 'NONE', *, *, #124215, .T. ) ;
#112297=CARTESIAN_POINT ( 'NONE',  ( -1.050000000000037792, 2.500000000000000000, 6.148780366869520009 ) ) ;
#112298=AXIS2_PLACEMENT_3D ( 'NONE', #116422, #26132, #88240 ) ;
#112299=AXIS2_PLACEMENT_3D ( 'NONE', #33296, #73204, #23449 ) ;
#112300=FACE_OUTER_BOUND ( 'NONE', #92838, .T. ) ;
#112301=ORIENTED_EDGE ( 'NONE', *, *, #27682, .F. ) ;
#112302=VERTEX_POINT ( 'NONE', #99620 ) ;
#112303=ORIENTED_EDGE ( 'NONE', *, *, #81101, .F. ) ;
#112304=DIRECTION ( 'NONE',  ( 0.000000000000000000, 0.000000000000000000, -1.000000000000000000 ) ) ;
#112305=DIRECTION ( 'NONE',  ( 0.000000000000000000, -0.9999939076577903929, 0.003490651415223739937 ) ) ;
#112307=CARTESIAN_POINT ( 'NONE',  ( -6.900000000000019007, 2.500000000000000000, -3.883716857408426648 ) ) ;
#112308=AXIS2_PLACEMENT_3D ( 'NONE', #64043, #54228, #42486 ) ;
#112309=CARTESIAN_POINT ( 'NONE',  ( 4.599999999999936584, 2.500000000000000000, 4.430127018922196847 ) ) ;
#112310=AXIS2_PLACEMENT_3D ( 'NONE', #20236, #80451, #68035 ) ;
#112312=EDGE_CURVE ( 'NONE', #125598, #51588, #103843, .T. ) ;
#112313=CARTESIAN_POINT ( 'NONE',  ( 21.24754738303277080, -0.7337760880902354232, 4.182111650399362723 ) ) ;
#112314=AXIS2_PLACEMENT_3D ( 'NONE', #15039, #94925, #115176 ) ;
#112315=CIRCLE ( 'NONE', #55862, 0.1000000000000002554 ) ;
#112316=CARTESIAN_POINT ( 'NONE',  ( -2.100000000000034728, 2.500000000000000000, 4.330127018922196314 ) ) ;
#112318=DIRECTION ( 'NONE',  ( 0.000000000000000000, 0.000000000000000000, -1.000000000000000000 ) ) ;
#112319=EDGE_CURVE ( 'NONE', #2580, #9598, #34909, .T. ) ;
#112320=CARTESIAN_POINT ( 'NONE',  ( 97.50000000000000000, 0.000000000000000000, 0.000000000000000000 ) ) ;
#112321=DIRECTION ( 'NONE',  ( 0.000000000000000000, 0.000000000000000000, 1.000000000000000000 ) ) ;
#112322=LINE ( 'NONE', #3648, #81507 ) ;
#112323=ORIENTED_EDGE ( 'NONE', *, *, #110626, .F. ) ;
#112324=DIRECTION ( 'NONE',  ( -0.000000000000000000, -1.000000000000000000, -0.000000000000000000 ) ) ;
#112325=AXIS2_PLACEMENT_3D ( 'NONE', #84049, #84703, #124634 ) ;
#112326=DIRECTION ( 'NONE',  ( 0.000000000000000000, 0.000000000000000000, 1.000000000000000000 ) ) ;
#112327=DIRECTION ( 'NONE',  ( 0.000000000000000000, 0.000000000000000000, -1.000000000000000000 ) ) ;
#112328=ORIENTED_EDGE ( 'NONE', *, *, #2863, .T. ) ;
#112329=VECTOR ( 'NONE', #80541, 1000.000000000000000 ) ;
#112331=AXIS2_PLACEMENT_3D ( 'NONE', #49575, #67225, #98640 ) ;
#112332=CARTESIAN_POINT ( 'NONE',  ( -11.44999999999999751, 12.50000000000000000, 1.818653347947321475 ) ) ;
#112334=ORIENTED_EDGE ( 'NONE', *, *, #103374, .T. ) ;
#112335=ORIENTED_EDGE ( 'NONE', *, *, #9310, .T. ) ;
#112336=CARTESIAN_POINT ( 'NONE',  ( 8.349999999999923261, 12.50000000000000000, 1.472243186433545459 ) ) ;
#112337=CONICAL_SURFACE ( 'NONE', #3664, 0.1000000000000000056, 0.003490658503988666988 ) ;
#112338=LINE ( 'NONE', #24600, #88615 ) ;
#112339=FACE_OUTER_BOUND ( 'NONE', #22139, .T. ) ;
#112340=AXIS2_PLACEMENT_3D ( 'NONE', #34493, #73111, #101282 ) ;
#112341=DIRECTION ( 'NONE',  ( 0.000000000000000000, 0.000000000000000000, -1.000000000000000000 ) ) ;
#112342=ORIENTED_EDGE ( 'NONE', *, *, #105907, .T. ) ;
#112343=AXIS2_PLACEMENT_3D ( 'NONE', #89907, #68979, #108888 ) ;
#112344=AXIS2_PLACEMENT_3D ( 'NONE', #77865, #127623, #37328 ) ;
#112345=EDGE_CURVE ( 'NONE', #28931, #58767, #41176, .T. ) ;
#112346=DIRECTION ( 'NONE',  ( 0.000000000000000000, 0.000000000000000000, 1.000000000000000000 ) ) ;
#112348=VERTEX_POINT ( 'NONE', #70158 ) ;
#112349=CARTESIAN_POINT ( 'NONE',  ( 16.64732342991096203, 0.5906619306577837181, 5.996708608299528009 ) ) ;
#112350=DIRECTION ( 'NONE',  ( 0.000000000000000000, 1.000000000000000000, 0.000000000000000000 ) ) ;
#112351=EDGE_CURVE ( 'NONE', #24119, #56014, #26572, .T. ) ;
#112352=EDGE_LOOP ( 'NONE', ( #128441, #9686 ) ) ;
#112353=AXIS2_PLACEMENT_3D ( 'NONE', #104504, #56042, #16747 ) ;
#112355=VERTEX_POINT ( 'NONE', #12507 ) ;
#112356=ORIENTED_EDGE ( 'NONE', *, *, #81243, .F. ) ;
#112357=CARTESIAN_POINT ( 'NONE',  ( 8.099999999999923261, 2.500000000000000000, 3.883716857408420431 ) ) ;
#112358=CARTESIAN_POINT ( 'NONE',  ( 14.37945523803923287, 1.499999999999936273, 7.667852710426877216 ) ) ;
#112359=EDGE_CURVE ( 'NONE', #74685, #41154, #41985, .T. ) ;
#112360=ADVANCED_FACE ( 'NONE', ( #110078 ), #105990, .T. ) ;
#112361=DIRECTION ( 'NONE',  ( -0.000000000000000000, -1.000000000000000000, -0.000000000000000000 ) ) ;
#112362=EDGE_CURVE ( 'NONE', #10740, #35393, #10565, .T. ) ;
#112363=FACE_BOUND ( 'NONE', #92692, .T. ) ;
#112365=ADVANCED_FACE ( 'NONE', ( #757 ), #7676, .T. ) ;
#112367=EDGE_CURVE ( 'NONE', #18925, #125929, #80866, .T. ) ;
#112368=DIRECTION ( 'NONE',  ( 0.000000000000000000, 0.000000000000000000, 1.000000000000000000 ) ) ;
#112369=DIRECTION ( 'NONE',  ( 0.000000000000000000, 0.000000000000000000, 1.000000000000000000 ) ) ;
#112370=CARTESIAN_POINT ( 'NONE',  ( -1.450000000000036371, 2.500000000000000000, 6.841600689897072485 ) ) ;
#112371=DIRECTION ( 'NONE',  ( -0.000000000000000000, 1.000000000000000000, -0.000000000000000000 ) ) ;
#112373=AXIS2_PLACEMENT_3D ( 'NONE', #28319, #97055, #68229 ) ;
#112374=EDGE_CURVE ( 'NONE', #119283, #8339, #15053, .T. ) ;
#112375=CARTESIAN_POINT ( 'NONE',  ( 2.299999999999949640, 2.500000000000000000, -4.676537180435977881 ) ) ;
#112376=ADVANCED_FACE ( 'NONE', ( #114567 ), #66274, .T. ) ;
#112377=EDGE_CURVE ( 'NONE', #90163, #101350, #68331, .T. ) ;
#112379=EDGE_LOOP ( 'NONE', ( #38250, #39422, #61666, #83285 ) ) ;
#112380=ORIENTED_EDGE ( 'NONE', *, *, #62258, .F. ) ;
#112381=VERTEX_POINT ( 'NONE', #13138 ) ;
#112382=ORIENTED_EDGE ( 'NONE', *, *, #55031, .F. ) ;
#112383=VERTEX_POINT ( 'NONE', #123119 ) ;
#112384=CARTESIAN_POINT ( 'NONE',  ( 4.599999999999940137, 12.50000000000000000, -5.022947341949754119 ) ) ;
#112385=CARTESIAN_POINT ( 'NONE',  ( 2.899999999999944844, 12.50000000000000000, 5.022947341949748790 ) ) ;
#112386=EDGE_LOOP ( 'NONE', ( #83723, #89821, #38318, #49475 ) ) ;
#112387=FACE_BOUND ( 'NONE', #2006, .T. ) ;
#112388=DIRECTION ( 'NONE',  ( 0.000000000000000000, -0.9999939076577903929, 0.003490651415223739937 ) ) ;
#112389=AXIS2_PLACEMENT_3D ( 'NONE', #108867, #108235, #88602 ) ;
#112390=AXIS2_PLACEMENT_3D ( 'NONE', #63064, #13951, #21868 ) ;
#112391=ORIENTED_EDGE ( 'NONE', *, *, #63750, .F. ) ;
#112392=CYLINDRICAL_SURFACE ( 'NONE', #20218, 2.000000000000000000 ) ;
#112393=DIRECTION ( 'NONE',  ( -0.000000000000000000, -1.000000000000000000, -0.000000000000000000 ) ) ;
#112394=LINE ( 'NONE', #84202, #91403 ) ;
#112395=EDGE_LOOP ( 'NONE', ( #48461, #127830 ) ) ;
#112396=CARTESIAN_POINT ( 'NONE',  ( -1.650000000000034328, 2.500000000000000000, -6.495190528383302464 ) ) ;
#112397=AXIS2_PLACEMENT_3D ( 'NONE', #108248, #18586, #66391 ) ;
#112398=ORIENTED_EDGE ( 'NONE', *, *, #98579, .T. ) ;
#112400=VECTOR ( 'NONE', #109942, 1000.000000000000000 ) ;
#112401=ORIENTED_EDGE ( 'NONE', *, *, #29022, .T. ) ;
#112402=VERTEX_POINT ( 'NONE', #64828 ) ;
#112403=CARTESIAN_POINT ( 'NONE',  ( -9.150000000000009237, 2.500000000000000000, 2.265063509461097357 ) ) ;
#112404=CARTESIAN_POINT ( 'NONE',  ( 1.649999999999950617, 2.500000000000000000, -2.265063509461101798 ) ) ;
#112405=CARTESIAN_POINT ( 'NONE',  ( -6.850000000000017408, 2.500000000000000000, -2.611473670974877592 ) ) ;
#112406=ORIENTED_EDGE ( 'NONE', *, *, #80415, .F. ) ;
#112407=CARTESIAN_POINT ( 'NONE',  ( -13.94999999999998685, 2.500000000000000000, -2.611473670974875372 ) ) ;
#112408=VECTOR ( 'NONE', #26905, 1000.000000000000000 ) ;
#112409=CARTESIAN_POINT ( 'NONE',  ( -11.05000000000000249, 2.500000000000000000, -1.818653347947322141 ) ) ;
#112410=FACE_OUTER_BOUND ( 'NONE', #80144, .T. ) ;
#112411=DIRECTION ( 'NONE',  ( 0.000000000000000000, 1.000000000000000000, 0.000000000000000000 ) ) ;
#112412=DIRECTION ( 'NONE',  ( 0.000000000000000000, 0.000000000000000000, 1.000000000000000000 ) ) ;
#112413=EDGE_LOOP ( 'NONE', ( #57630, #2645 ) ) ;
#112414=CONICAL_SURFACE ( 'NONE', #7935, 0.09999999999999982514, 0.003490658503988666988 ) ;
#112415=FACE_OUTER_BOUND ( 'NONE', #4499, .T. ) ;
#112416=ADVANCED_FACE ( 'NONE', ( #32822 ), #28634, .T. ) ;
#112417=ORIENTED_EDGE ( 'NONE', *, *, #96325, .T. ) ;
#112418=CARTESIAN_POINT ( 'NONE',  ( 9.799999999999915445, 12.50000000000000000, 3.918623584224383727 ) ) ;
#112419=EDGE_CURVE ( 'NONE', #79956, #27779, #43285, .T. ) ;
#112420=CIRCLE ( 'NONE', #55963, 0.06509327318403745899 ) ;
#112421=EDGE_LOOP ( 'NONE', ( #11094, #86343 ) ) ;
#112422=EDGE_CURVE ( 'NONE', #38146, #96104, #11988, .T. ) ;
#112423=VERTEX_POINT ( 'NONE', #4588 ) ;
#112424=DIRECTION ( 'NONE',  ( 0.000000000000000000, 1.000000000000000000, 0.000000000000000000 ) ) ;
#112425=VECTOR ( 'NONE', #25805, 1000.000000000000000 ) ;
#112426=CARTESIAN_POINT ( 'NONE',  ( 2.899999999999946620, 12.50000000000000000, -4.957854068765716882 ) ) ;
#112427=CARTESIAN_POINT ( 'NONE',  ( 3.099999999999945022, 2.500000000000000000, -0.3464101615137783474 ) ) ;
#112428=DIRECTION ( 'NONE',  ( 0.000000000000000000, 1.000000000000000000, 0.000000000000000000 ) ) ;
#112429=PLANE ( 'NONE',  #14065 ) ;
#112430=CIRCLE ( 'NONE', #24587, 0.1000000000000000472 ) ;
#112431=ORIENTED_EDGE ( 'NONE', *, *, #92914, .F. ) ;
#112432=AXIS2_PLACEMENT_3D ( 'NONE', #70092, #78639, #68794 ) ;
#112433=ADVANCED_FACE ( 'NONE', ( #112655 ), #97669, .T. ) ;
#112434=ORIENTED_EDGE ( 'NONE', *, *, #60972, .T. ) ;
#112435=FACE_OUTER_BOUND ( 'NONE', #114855, .T. ) ;
#112436=AXIS2_PLACEMENT_3D ( 'NONE', #125843, #123281, #6061 ) ;
#112437=CARTESIAN_POINT ( 'NONE',  ( 10.84999999999991260, 2.500000000000000000, 5.702370205355745014 ) ) ;
#112438=CARTESIAN_POINT ( 'NONE',  ( -10.85000000000000142, 2.500000000000000000, -7.188010851410850499 ) ) ;
#112439=ORIENTED_EDGE ( 'NONE', *, *, #110364, .F. ) ;
#112441=CARTESIAN_POINT ( 'NONE',  ( -6.050000000000022027, 2.500000000000000000, -6.148780366869526226 ) ) ;
#112442=AXIS2_PLACEMENT_3D ( 'NONE', #10015, #60428, #91154 ) ;
#112443=CIRCLE ( 'NONE', #74582, 0.06509327318403745899 ) ;
#112444=EDGE_LOOP ( 'NONE', ( #11561, #54671 ) ) ;
#112445=CARTESIAN_POINT ( 'NONE',  ( -6.700000000000019718, 2.500000000000000000, -0.1000000000000023925 ) ) ;
#112446=CARTESIAN_POINT ( 'NONE',  ( -13.09999999999999254, 2.500000000000000000, -4.576537180435974683 ) ) ;
#112447=AXIS2_PLACEMENT_3D ( 'NONE', #23471, #94792, #92203 ) ;
#112448=CARTESIAN_POINT ( 'NONE',  ( 0.3999999999999555023, 2.500000000000000000, 4.230127018922196669 ) ) ;
#112449=ORIENTED_EDGE ( 'NONE', *, *, #42404, .F. ) ;
#112450=DIRECTION ( 'NONE',  ( 0.000000000000000000, -0.000000000000000000, 1.000000000000000000 ) ) ;
#112451=DIRECTION ( 'NONE',  ( 0.000000000000000000, 1.000000000000000000, 0.000000000000000000 ) ) ;
#112452=PLANE ( 'NONE',  #35780 ) ;
#112453=CARTESIAN_POINT ( 'NONE',  ( -14.99999999999998224, 2.500000000000000000, -0.7928203230275518987 ) ) ;
#112454=CONICAL_SURFACE ( 'NONE', #58069, 0.09999999999999982514, 0.003490658503988666988 ) ;
#112455=ADVANCED_FACE ( 'NONE', ( #15722 ), #60138, .T. ) ;
#112456=DIRECTION ( 'NONE',  ( 0.000000000000000000, 1.000000000000000000, 0.000000000000000000 ) ) ;
#112457=VERTEX_POINT ( 'NONE', #123736 ) ;
#112458=DIRECTION ( 'NONE',  ( 0.000000000000000000, 0.000000000000000000, -1.000000000000000000 ) ) ;
#112459=AXIS2_PLACEMENT_3D ( 'NONE', #85233, #6629, #35503 ) ;
#112460=CONICAL_SURFACE ( 'NONE', #72737, 0.1000000000000002554, 0.003490658503988666988 ) ;
#112461=DIRECTION ( 'NONE',  ( -0.000000000000000000, 1.000000000000000000, -0.000000000000000000 ) ) ;
#112462=ORIENTED_EDGE ( 'NONE', *, *, #84833, .T. ) ;
#112463=VERTEX_POINT ( 'NONE', #54369 ) ;
#112465=DIRECTION ( 'NONE',  ( 0.000000000000000000, -0.9999939076577903929, 0.003490651415223739937 ) ) ;
#112466=CARTESIAN_POINT ( 'NONE',  ( 5.199999999999933564, 2.500000000000000000, 3.983716857408420076 ) ) ;
#112467=CARTESIAN_POINT ( 'NONE',  ( -5.450000000000023270, 2.500000000000000000, -6.495190528383302464 ) ) ;
#112468=CARTESIAN_POINT ( 'NONE',  ( 4.599999999999936584, 12.50000000000000000, 3.702399969078682407 ) ) ;
#112469=FACE_OUTER_BOUND ( 'NONE', #110306, .T. ) ;
#112470=EDGE_CURVE ( 'NONE', #17072, #64922, #37138, .T. ) ;
#112471=FACE_OUTER_BOUND ( 'NONE', #106658, .T. ) ;
#112472=CARTESIAN_POINT ( 'NONE',  ( 11.84999999999990727, 2.500000000000000000, 6.048780366869520364 ) ) ;
#112473=CARTESIAN_POINT ( 'NONE',  ( -0.8500000000000386136, 2.500000000000000000, 2.857883832488649301 ) ) ;
#112475=ORIENTED_EDGE ( 'NONE', *, *, #54300, .T. ) ;
#112476=ORIENTED_EDGE ( 'NONE', *, *, #80475, .F. ) ;
#112477=VECTOR ( 'NONE', #19498, 1000.000000000000000 ) ;
#112478=ORIENTED_EDGE ( 'NONE', *, *, #118703, .F. ) ;
#112479=EDGE_CURVE ( 'NONE', #122530, #78195, #33463, .T. ) ;
#112480=FACE_OUTER_BOUND ( 'NONE', #76338, .T. ) ;
#112481=CARTESIAN_POINT ( 'NONE',  ( 5.849999999999935696, 12.50000000000000000, -6.495190528383302464 ) ) ;
#112482=ORIENTED_EDGE ( 'NONE', *, *, #44667, .T. ) ;
#112484=CIRCLE ( 'NONE', #127062, 0.1000000000000002554 ) ;
#112485=DIRECTION ( 'NONE',  ( 0.000000000000000000, 0.000000000000000000, 1.000000000000000000 ) ) ;
#112486=DIRECTION ( 'NONE',  ( 0.000000000000000000, 1.000000000000000000, 0.000000000000000000 ) ) ;
#112487=ORIENTED_EDGE ( 'NONE', *, *, #36152, .T. ) ;
#112488=ADVANCED_FACE ( 'NONE', ( #94955 ), #47505, .T. ) ;
#112489=DIRECTION ( 'NONE',  ( 0.000000000000000000, 0.000000000000000000, -1.000000000000000000 ) ) ;
#112490=CIRCLE ( 'NONE', #129143, 0.06509327318403743123 ) ;
#112491=LINE ( 'NONE', #53567, #62579 ) ;
#112492=ORIENTED_EDGE ( 'NONE', *, *, #82069, .F. ) ;
#112493=CONICAL_SURFACE ( 'NONE', #33091, 0.1000000000000000056, 0.003490658503988666988 ) ;
#112494=ORIENTED_EDGE ( 'NONE', *, *, #122704, .T. ) ;
#112495=VERTEX_POINT ( 'NONE', #105412 ) ;
#112496=VERTEX_POINT ( 'NONE', #44557 ) ;
#112497=DIRECTION ( 'NONE',  ( -0.000000000000000000, -1.000000000000000000, -0.000000000000000000 ) ) ;
#112498=LINE ( 'NONE', #31366, #82272 ) ;
#112499=CARTESIAN_POINT ( 'NONE',  ( -2.100000000000033396, 2.500000000000000000, -0.6928203230275542523 ) ) ;
#112500=CARTESIAN_POINT ( 'NONE',  ( -15.59999999999998010, 2.500000000000000000, -0.3464101615137759604 ) ) ;
#112501=AXIS2_PLACEMENT_3D ( 'NONE', #29488, #60254, #73269 ) ;
#112502=ORIENTED_EDGE ( 'NONE', *, *, #75338, .F. ) ;
#112503=EDGE_CURVE ( 'NONE', #116053, #80727, #3671, .T. ) ;
#112504=CARTESIAN_POINT ( 'NONE',  ( -0.6500000000000394351, 2.500000000000000000, 2.411473670974873862 ) ) ;
#112505=ORIENTED_EDGE ( 'NONE', *, *, #16992, .T. ) ;
#112506=CIRCLE ( 'NONE', #114630, 0.1000000000000002554 ) ;
#112507=DIRECTION ( 'NONE',  ( -4.274815082592931898E-19, -0.9999939076577903929, -0.003490651415223739937 ) ) ;
#112508=CARTESIAN_POINT ( 'NONE',  ( 4.912722231824926844, -1.499999999999620082, -9.942384337864403676 ) ) ;
#112509=DIRECTION ( 'NONE',  ( -0.000000000000000000, -1.000000000000000000, -0.000000000000000000 ) ) ;
#112510=CARTESIAN_POINT ( 'NONE',  ( 4.599999999999936584, 12.50000000000000000, 4.330127018922196314 ) ) ;
#112511=ADVANCED_FACE ( 'NONE', ( #23623 ), #24518, .T. ) ;
#112512=VERTEX_POINT ( 'NONE', #125040 ) ;
#112513=AXIS2_PLACEMENT_3D ( 'NONE', #66720, #106654, #59524 ) ;
#112514=ORIENTED_EDGE ( 'NONE', *, *, #24584, .T. ) ;
#112515=ORIENTED_EDGE ( 'NONE', *, *, #97288, .T. ) ;
#112516=DIRECTION ( 'NONE',  ( -0.000000000000000000, 1.000000000000000000, -0.000000000000000000 ) ) ;
#112517=CARTESIAN_POINT ( 'NONE',  ( 6.249999999999930722, 12.50000000000000000, -1.537336459617587581 ) ) ;
#112518=EDGE_CURVE ( 'NONE', #76477, #80752, #114387, .T. ) ;
#112519=EDGE_CURVE ( 'NONE', #67433, #112003, #106082, .T. ) ;
#112520=DIRECTION ( 'NONE',  ( -0.000000000000000000, 1.000000000000000000, -0.000000000000000000 ) ) ;
#112521=EDGE_CURVE ( 'NONE', #54360, #1523, #87194, .T. ) ;
#112522=FACE_BOUND ( 'NONE', #50819, .T. ) ;
#112523=AXIS2_PLACEMENT_3D ( 'NONE', #111094, #21450, #106928 ) ;
#112524=ADVANCED_FACE ( 'NONE', ( #86397 ), #17661, .T. ) ;
#112525=CARTESIAN_POINT ( 'NONE',  ( 12.94999999999989981, 2.500000000000000000, -2.165063509461101710 ) ) ;
#112526=CARTESIAN_POINT ( 'NONE',  ( 8.949999999999921130, 12.50000000000000000, 1.818653347947321475 ) ) ;
#112527=AXIS2_PLACEMENT_3D ( 'NONE', #12124, #52075, #120801 ) ;
#112528=DIRECTION ( 'NONE',  ( 0.000000000000000000, 0.000000000000000000, 1.000000000000000000 ) ) ;
#112529=AXIS2_PLACEMENT_3D ( 'NONE', #119900, #71423, #60973 ) ;
#112530=EDGE_CURVE ( 'NONE', #126433, #54302, #18942, .T. ) ;
#112531=CARTESIAN_POINT ( 'NONE',  ( -12.89999999999999325, 12.50000000000000000, -3.572213422710609709 ) ) ;
#112532=ADVANCED_FACE ( 'NONE', ( #128286 ), #85754, .T. ) ;
#112533=AXIS2_PLACEMENT_3D ( 'NONE', #86476, #56371, #126413 ) ;
#112534=CARTESIAN_POINT ( 'NONE',  ( -8.350000000000010303, 2.500000000000000000, 6.595190528383296780 ) ) ;
#112535=EDGE_CURVE ( 'NONE', #75419, #30036, #89360, .T. ) ;
#112536=DIRECTION ( 'NONE',  ( 0.000000000000000000, -0.9999939076577903929, 0.003490651415223739937 ) ) ;
#112537=EDGE_LOOP ( 'NONE', ( #93124, #79744 ) ) ;
#112538=EDGE_CURVE ( 'NONE', #12633, #81499, #76846, .T. ) ;
#112540=DIRECTION ( 'NONE',  ( 0.000000000000000000, 0.000000000000000000, -1.000000000000000000 ) ) ;
#112542=ORIENTED_EDGE ( 'NONE', *, *, #117045, .T. ) ;
#112543=CARTESIAN_POINT ( 'NONE',  ( -8.550000000000009592, 12.50000000000000000, 6.841600689897072485 ) ) ;
#112544=CIRCLE ( 'NONE', #116720, 0.1000000000000002554 ) ;
#112545=DIRECTION ( 'NONE',  ( 0.000000000000000000, 0.000000000000000000, 1.000000000000000000 ) ) ;
#112546=FACE_BOUND ( 'NONE', #108906, .T. ) ;
#112547=ADVANCED_FACE ( 'NONE', ( #125673 ), #49669, .T. ) ;
#112548=DIRECTION ( 'NONE',  ( 0.000000000000000000, 0.000000000000000000, 1.000000000000000000 ) ) ;
#112550=AXIS2_PLACEMENT_3D ( 'NONE', #83832, #83212, #123748 ) ;
#112551=ORIENTED_EDGE ( 'NONE', *, *, #114870, .T. ) ;
#112553=DIRECTION ( 'NONE',  ( -0.000000000000000000, 1.000000000000000000, -0.000000000000000000 ) ) ;
#112554=ORIENTED_EDGE ( 'NONE', *, *, #54866, .T. ) ;
#112555=FACE_OUTER_BOUND ( 'NONE', #72357, .T. ) ;
#112556=CARTESIAN_POINT ( 'NONE',  ( 8.349999999999923261, 2.500000000000000000, -5.802370205355749988 ) ) ;
#112557=VERTEX_POINT ( 'NONE', #76591 ) ;
#112558=AXIS2_PLACEMENT_3D ( 'NONE', #30133, #102080, #62167 ) ;
#112559=LINE ( 'NONE', #109975, #38114 ) ;
#112560=CARTESIAN_POINT ( 'NONE',  ( 13.74999999999993072, 2.500000000000000000, -2.165063509461101710 ) ) ;
#112561=ORIENTED_EDGE ( 'NONE', *, *, #98279, .F. ) ;
#112562=CONICAL_SURFACE ( 'NONE', #79122, 0.1000000000000002554, 0.003490658503988666988 ) ;
#112563=DIRECTION ( 'NONE',  ( -4.274815082592931898E-19, -0.9999939076577903929, -0.003490651415223739937 ) ) ;
#112564=CIRCLE ( 'NONE', #50161, 0.06509327318403745899 ) ;
#112566=AXIS2_PLACEMENT_3D ( 'NONE', #12280, #41782, #50949 ) ;
#112567=CARTESIAN_POINT ( 'NONE',  ( 11.44999999999990870, 2.500000000000000000, 6.941600689897073018 ) ) ;
#112568=ORIENTED_EDGE ( 'NONE', *, *, #49195, .F. ) ;
#112569=VERTEX_POINT ( 'NONE', #57606 ) ;
#112571=AXIS2_PLACEMENT_3D ( 'NONE', #31767, #120778, #101796 ) ;
#112572=VERTEX_POINT ( 'NONE', #97513 ) ;
#112573=DIRECTION ( 'NONE',  ( 0.000000000000000000, 0.000000000000000000, -1.000000000000000000 ) ) ;
#112574=DIRECTION ( 'NONE',  ( 0.000000000000000000, 0.000000000000000000, 1.000000000000000000 ) ) ;
#112575=ADVANCED_FACE ( 'NONE', ( #45847 ), #1518, .T. ) ;
#112576=CONICAL_SURFACE ( 'NONE', #22698, 0.1000000000000002554, 0.003490658503988666988 ) ;
#112577=ORIENTED_EDGE ( 'NONE', *, *, #2709, .F. ) ;
#112578=DIRECTION ( 'NONE',  ( 0.000000000000000000, 0.000000000000000000, 1.000000000000000000 ) ) ;
#112579=EDGE_CURVE ( 'NONE', #93656, #83109, #115868, .T. ) ;
#112580=DIRECTION ( 'NONE',  ( 0.000000000000000000, 0.000000000000000000, -1.000000000000000000 ) ) ;
#112581=FACE_OUTER_BOUND ( 'NONE', #44750, .T. ) ;
#112582=DIRECTION ( 'NONE',  ( 0.000000000000000000, 1.000000000000000000, 0.000000000000000000 ) ) ;
#112583=CARTESIAN_POINT ( 'NONE',  ( -6.650000000000014566, 2.500000000000000000, 2.065063509461097624 ) ) ;
#112584=CONICAL_SURFACE ( 'NONE', #56123, 0.1000000000000000472, 0.003490658503988666988 ) ;
#112585=EDGE_CURVE ( 'NONE', #70628, #73131, #16351, .T. ) ;
#112586=ORIENTED_EDGE ( 'NONE', *, *, #126262, .T. ) ;
#112587=CONICAL_SURFACE ( 'NONE', #1750, 0.1000000000000002554, 0.003490658503988666988 ) ;
#112588=EDGE_LOOP ( 'NONE', ( #41438, #82057, #25684, #56199 ) ) ;
#112589=CARTESIAN_POINT ( 'NONE',  ( -1.250000000000001554, 2.500000000000000000, 2.165063509461097713 ) ) ;
#112590=VERTEX_POINT ( 'NONE', #7838 ) ;
#112591=DIRECTION ( 'NONE',  ( 0.000000000000000000, -0.9999939076577903929, 0.003490651415223739937 ) ) ;
#112592=ORIENTED_EDGE ( 'NONE', *, *, #26689, .T. ) ;
#112593=VERTEX_POINT ( 'NONE', #7190 ) ;
#112594=EDGE_LOOP ( 'NONE', ( #23026, #41196 ) ) ;
#112595=DIRECTION ( 'NONE',  ( 0.000000000000000000, 1.000000000000000000, 0.000000000000000000 ) ) ;
#112596=CARTESIAN_POINT ( 'NONE',  ( 12.89999999999989910, 12.50000000000000000, 0.6928203230275494784 ) ) ;
#112597=DIRECTION ( 'NONE',  ( 0.000000000000000000, 0.000000000000000000, -1.000000000000000000 ) ) ;
#112598=CARTESIAN_POINT ( 'NONE',  ( 105.5000000000000142, 0.000000000000000000, 0.000000000000000000 ) ) ;
#112601=LINE ( 'NONE', #13077, #25555 ) ;
#112602=PLANE ( 'NONE',  #103511 ) ;
#112603=CIRCLE ( 'NONE', #77085, 0.1000000000000002554 ) ;
#112604=DIRECTION ( 'NONE',  ( -0.000000000000000000, -1.000000000000000000, -0.000000000000000000 ) ) ;
#112605=LINE ( 'NONE', #31466, #24739 ) ;
#112606=AXIS2_PLACEMENT_3D ( 'NONE', #64642, #35203, #13599 ) ;
#112607=ORIENTED_EDGE ( 'NONE', *, *, #65260, .T. ) ;
#112608=DIRECTION ( 'NONE',  ( 0.000000000000000000, 1.000000000000000000, 0.000000000000000000 ) ) ;
#112609=VERTEX_POINT ( 'NONE', #78548 ) ;
#112610=ORIENTED_EDGE ( 'NONE', *, *, #78276, .T. ) ;
#112611=DIRECTION ( 'NONE',  ( 0.000000000000000000, 0.000000000000000000, 1.000000000000000000 ) ) ;
#112612=CARTESIAN_POINT ( 'NONE',  ( 8.299999999999922551, 12.50000000000000000, -4.330127018922201643 ) ) ;
#112613=CONICAL_SURFACE ( 'NONE', #100090, 0.09999999999999982514, 0.003490658503988666988 ) ;
#112614=DIRECTION ( 'NONE',  ( 0.000000000000000000, 0.000000000000000000, 1.000000000000000000 ) ) ;
#112615=EDGE_CURVE ( 'NONE', #45445, #29934, #53755, .T. ) ;
#112616=DIRECTION ( 'NONE',  ( 0.000000000000000000, 0.000000000000000000, -1.000000000000000000 ) ) ;
#112618=DIRECTION ( 'NONE',  ( 0.000000000000000000, 1.000000000000000000, 0.000000000000000000 ) ) ;
#112619=LINE ( 'NONE', #54333, #15575 ) ;
#112620=CARTESIAN_POINT ( 'NONE',  ( 11.64999999999990798, 2.500000000000000000, -2.957883832488653830 ) ) ;
#112621=EDGE_LOOP ( 'NONE', ( #126171, #4920, #117869, #8468 ) ) ;
#112622=AXIS2_PLACEMENT_3D ( 'NONE', #73425, #113355, #81960 ) ;
#112623=ORIENTED_EDGE ( 'NONE', *, *, #40594, .T. ) ;
#112624=VERTEX_POINT ( 'NONE', #126986 ) ;
#112625=CIRCLE ( 'NONE', #56166, 0.1000000000000002554 ) ;
#112626=EDGE_LOOP ( 'NONE', ( #56828, #90343 ) ) ;
#112627=EDGE_CURVE ( 'NONE', #115877, #71057, #116535, .T. ) ;
#112628=VECTOR ( 'NONE', #10313, 1000.000000000000000 ) ;
#112629=ADVANCED_FACE ( 'NONE', ( #87044 ), #55900, .T. ) ;
#112630=ORIENTED_EDGE ( 'NONE', *, *, #77646, .F. ) ;
#112631=DIRECTION ( 'NONE',  ( 0.000000000000000000, 1.000000000000000000, 0.000000000000000000 ) ) ;
#112632=FACE_OUTER_BOUND ( 'NONE', #90889, .T. ) ;
#112633=AXIS2_PLACEMENT_3D ( 'NONE', #100060, #69959, #39870 ) ;
#112634=CIRCLE ( 'NONE', #41542, 0.09999999999999999167 ) ;
#112635=DIRECTION ( 'NONE',  ( 0.000000000000000000, 0.000000000000000000, 1.000000000000000000 ) ) ;
#112636=FACE_OUTER_BOUND ( 'NONE', #41380, .T. ) ;
#112637=CARTESIAN_POINT ( 'NONE',  ( 9.199999999999919353, 2.500000000000000000, -2.276824562219559311E-15 ) ) ;
#112638=ORIENTED_EDGE ( 'NONE', *, *, #30277, .F. ) ;
#112639=CARTESIAN_POINT ( 'NONE',  ( 7.499999999999925393, 12.50000000000000000, 5.022947341949748790 ) ) ;
#112640=EDGE_CURVE ( 'NONE', #8229, #38593, #18246, .T. ) ;
#112641=CARTESIAN_POINT ( 'NONE',  ( -10.00000000000000711, 12.50000000000000000, -3.637306695894645614 ) ) ;
#112642=CARTESIAN_POINT ( 'NONE',  ( 14.99999999999989342, 12.50000000000000000, -0.7579135962115916003 ) ) ;
#112643=DIRECTION ( 'NONE',  ( 1.000000000000000000, 0.000000000000000000, 0.000000000000000000 ) ) ;
#112644=ORIENTED_EDGE ( 'NONE', *, *, #116075, .F. ) ;
#112646=VERTEX_POINT ( 'NONE', #68054 ) ;
#112647=AXIS2_PLACEMENT_3D ( 'NONE', #87577, #15610, #98049 ) ;
#112648=DIRECTION ( 'NONE',  ( 0.000000000000000000, -0.000000000000000000, 1.000000000000000000 ) ) ;
#112649=CARTESIAN_POINT ( 'NONE',  ( -1.050000000000038680, 2.500000000000000000, 2.611473670974873151 ) ) ;
#112650=LINE ( 'NONE', #62903, #37734 ) ;
#112651=CONICAL_SURFACE ( 'NONE', #49979, 0.1000000000000002554, 0.003490658503988666988 ) ;
#112652=AXIS2_PLACEMENT_3D ( 'NONE', #99750, #100385, #231 ) ;
#112653=ORIENTED_EDGE ( 'NONE', *, *, #62863, .F. ) ;
#112654=CARTESIAN_POINT ( 'NONE',  ( -6.650000000000014566, 2.500000000000000000, 6.395190528383296602 ) ) ;
#112655=FACE_OUTER_BOUND ( 'NONE', #4025, .T. ) ;
#112656=LINE ( 'NONE', #63562, #6514 ) ;
#112657=CARTESIAN_POINT ( 'NONE',  ( -2.499999999999996447, 12.50000000000000000, 4.265033745738159077 ) ) ;
#112658=AXIS2_PLACEMENT_3D ( 'NONE', #40192, #90567, #80115 ) ;
#112659=AXIS2_PLACEMENT_3D ( 'NONE', #86995, #7786, #98738 ) ;
#112660=EDGE_CURVE ( 'NONE', #10182, #18164, #58255, .T. ) ;
#112661=AXIS2_PLACEMENT_3D ( 'NONE', #46259, #96632, #35806 ) ;
#112662=CARTESIAN_POINT ( 'NONE',  ( 4.399999999999940847, 12.50000000000000000, -4.676537180435977881 ) ) ;
#112663=ORIENTED_EDGE ( 'NONE', *, *, #107782, .F. ) ;
#112664=ORIENTED_EDGE ( 'NONE', *, *, #117003, .F. ) ;
#112665=EDGE_CURVE ( 'NONE', #66158, #62754, #81117, .T. ) ;
#112667=DIRECTION ( 'NONE',  ( 0.000000000000000000, -0.9999939076577903929, 0.003490651415223739937 ) ) ;
#112668=CIRCLE ( 'NONE', #120986, 0.1000000000000002554 ) ;
#112669=EDGE_CURVE ( 'NONE', #51184, #37790, #124868, .T. ) ;
#112670=CARTESIAN_POINT ( 'NONE',  ( -12.04999999999999538, 2.500000000000000000, 2.265063509461097357 ) ) ;
#112671=DIRECTION ( 'NONE',  ( 0.000000000000000000, -0.9999939076577903929, 0.003490651415223739937 ) ) ;
#112672=CIRCLE ( 'NONE', #56219, 0.06509327318403745899 ) ;
#112673=ORIENTED_EDGE ( 'NONE', *, *, #109998, .F. ) ;
#112674=ADVANCED_FACE ( 'NONE', ( #61485 ), #79187, .T. ) ;
#112675=ADVANCED_FACE ( 'NONE', ( #91569 ), #45462, .T. ) ;
#112676=VERTEX_POINT ( 'NONE', #60195 ) ;
#112677=DIRECTION ( 'NONE',  ( 0.000000000000000000, -0.000000000000000000, 1.000000000000000000 ) ) ;
#112678=CARTESIAN_POINT ( 'NONE',  ( 2.949999999999946887, 12.50000000000000000, -6.495190528383302464 ) ) ;
#112679=EDGE_CURVE ( 'NONE', #93582, #59583, #62181, .T. ) ;
#112680=CARTESIAN_POINT ( 'NONE',  ( 3.349999999999945466, 2.500000000000000000, -2.165063509461101710 ) ) ;
#112681=DIRECTION ( 'NONE',  ( 0.000000000000000000, 0.000000000000000000, -1.000000000000000000 ) ) ;
#112682=ORIENTED_EDGE ( 'NONE', *, *, #74352, .F. ) ;
#112683=AXIS2_PLACEMENT_3D ( 'NONE', #57846, #10026, #66988 ) ;
#112684=DIRECTION ( 'NONE',  ( 0.000000000000000000, 1.000000000000000000, 0.000000000000000000 ) ) ;
#112685=ADVANCED_FACE ( 'NONE', ( #29435 ), #99832, .T. ) ;
#112686=PLANE ( 'NONE',  #82890 ) ;
#112687=AXIS2_PLACEMENT_3D ( 'NONE', #105872, #55486, #85582 ) ;
#112688=VERTEX_POINT ( 'NONE', #99469 ) ;
#112689=CARTESIAN_POINT ( 'NONE',  ( 4.149999999999938183, 12.50000000000000000, 7.253104124594885960 ) ) ;
#112690=EDGE_LOOP ( 'NONE', ( #55160, #27250 ) ) ;
#112691=EDGE_CURVE ( 'NONE', #34777, #9531, #83105, .T. ) ;
#112692=FACE_OUTER_BOUND ( 'NONE', #88170, .T. ) ;
#112693=ORIENTED_EDGE ( 'NONE', *, *, #42513, .T. ) ;
#112694=CONICAL_SURFACE ( 'NONE', #56248, 0.09999999999999982514, 0.003490658503988666988 ) ;
#112695=DIRECTION ( 'NONE',  ( 0.000000000000000000, 0.000000000000000000, -1.000000000000000000 ) ) ;
#112696=CARTESIAN_POINT ( 'NONE',  ( 1.649999999999951505, 2.500000000000000000, 2.957883832488649389 ) ) ;
#112697=ORIENTED_EDGE ( 'NONE', *, *, #69353, .T. ) ;
#112698=ORIENTED_EDGE ( 'NONE', *, *, #50755, .T. ) ;
#112700=FACE_OUTER_BOUND ( 'NONE', #58418, .T. ) ;
#112701=CONICAL_SURFACE ( 'NONE', #56156, 0.1000000000000002554, 0.003490658503988666988 ) ;
#112702=CARTESIAN_POINT ( 'NONE',  ( 6.849999999999929479, 2.500000000000000000, 6.148780366869520009 ) ) ;
#112704=VECTOR ( 'NONE', #70011, 1000.000000000000000 ) ;
#112705=DIRECTION ( 'NONE',  ( 0.000000000000000000, 0.000000000000000000, 1.000000000000000000 ) ) ;
#112706=FACE_OUTER_BOUND ( 'NONE', #127096, .T. ) ;
#112707=CARTESIAN_POINT ( 'NONE',  ( 2.499999999999948930, 12.50000000000000000, -4.957854068765716882 ) ) ;
#112708=CARTESIAN_POINT ( 'NONE',  ( 6.649999999999929301, 12.50000000000000000, 6.495190528383297135 ) ) ;
#112709=CARTESIAN_POINT ( 'NONE',  ( 14.39999999999989555, 2.500000000000000000, 0.3464101615137736845 ) ) ;
#112710=AXIS2_PLACEMENT_3D ( 'NONE', #111608, #103733, #45465 ) ;
#112711=ORIENTED_EDGE ( 'NONE', *, *, #42330, .F. ) ;
#112712=ORIENTED_EDGE ( 'NONE', *, *, #5829, .T. ) ;
#112713=CARTESIAN_POINT ( 'NONE',  ( 6.449999999999931788, 12.50000000000000000, -2.511473670974877948 ) ) ;
#112714=CONICAL_SURFACE ( 'NONE', #93838, 0.09999999999999999167, 0.003490658503988666988 ) ;
#112715=AXIS2_PLACEMENT_3D ( 'NONE', #40581, #51677, #19626 ) ;
#112716=EDGE_LOOP ( 'NONE', ( #4411, #51713 ) ) ;
#112718=DIRECTION ( 'NONE',  ( 0.000000000000000000, 1.000000000000000000, 0.000000000000000000 ) ) ;
#112719=FACE_OUTER_BOUND ( 'NONE', #8701, .T. ) ;
#112720=AXIS2_PLACEMENT_3D ( 'NONE', #21259, #9518, #981 ) ;
#112721=ORIENTED_EDGE ( 'NONE', *, *, #109089, .F. ) ;
#112722=ORIENTED_EDGE ( 'NONE', *, *, #88239, .T. ) ;
#112723=FACE_BOUND ( 'NONE', #45534, .T. ) ;
#112724=ORIENTED_EDGE ( 'NONE', *, *, #4997, .F. ) ;
#112725=DIRECTION ( 'NONE',  ( -0.000000000000000000, 1.000000000000000000, -0.000000000000000000 ) ) ;
#112726=CARTESIAN_POINT ( 'NONE',  ( -7.300000000000013145, 12.50000000000000000, 3.983716857408420076 ) ) ;
#112727=CARTESIAN_POINT ( 'NONE',  ( -3.150000000000029221, 12.50000000000000000, 2.511473670974873507 ) ) ;
#112728=CIRCLE ( 'NONE', #77124, 0.09999999999999982514 ) ;
#112729=CONICAL_SURFACE ( 'NONE', #56275, 0.1000000000000002554, 0.003490658503988666988 ) ;
#112730=CARTESIAN_POINT ( 'NONE',  ( -0.8500000000000395017, 2.500000000000000000, 2.165063509461097713 ) ) ;
#112731=EDGE_CURVE ( 'NONE', #33136, #19384, #114478, .T. ) ;
#112732=DIRECTION ( 'NONE',  ( 0.000000000000000000, 0.000000000000000000, 1.000000000000000000 ) ) ;
#112733=DIRECTION ( 'NONE',  ( 0.000000000000000000, 0.000000000000000000, 1.000000000000000000 ) ) ;
#112734=DIRECTION ( 'NONE',  ( -0.000000000000000000, -1.000000000000000000, -0.000000000000000000 ) ) ;
#112735=CARTESIAN_POINT ( 'NONE',  ( -15.19999999999998153, 2.500000000000000000, -0.2464101615137759549 ) ) ;
#112736=DIRECTION ( 'NONE',  ( -0.000000000000000000, -1.000000000000000000, -0.000000000000000000 ) ) ;
#112737=LINE ( 'NONE', #121259, #127893 ) ;
#112738=DIRECTION ( 'NONE',  ( -0.000000000000000000, -1.000000000000000000, -0.000000000000000000 ) ) ;
#112739=EDGE_CURVE ( 'NONE', #30668, #119878, #82374, .T. ) ;
#112740=ORIENTED_EDGE ( 'NONE', *, *, #119028, .T. ) ;
#112741=EDGE_LOOP ( 'NONE', ( #16903, #81301 ) ) ;
#112742=VERTEX_POINT ( 'NONE', #79811 ) ;
#112743=CARTESIAN_POINT ( 'NONE',  ( 10.84999999999991260, 2.500000000000000000, 5.802370205355744659 ) ) ;
#112744=ORIENTED_EDGE ( 'NONE', *, *, #102174, .T. ) ;
#112745=CONICAL_SURFACE ( 'NONE', #29127, 0.1000000000000002554, 0.003490658503988666988 ) ;
#112746=CARTESIAN_POINT ( 'NONE',  ( -0.4000000000000392131, 2.500000000000000000, -5.022947341949754119 ) ) ;
#112747=EDGE_LOOP ( 'NONE', ( #81672, #104213 ) ) ;
#112748=EDGE_LOOP ( 'NONE', ( #61449, #59925 ) ) ;
#112749=ORIENTED_EDGE ( 'NONE', *, *, #52360, .T. ) ;
#112750=FACE_OUTER_BOUND ( 'NONE', #67468, .T. ) ;
#112751=CONICAL_SURFACE ( 'NONE', #110673, 0.09999999999999982514, 0.003490658503988666988 ) ;
#112752=AXIS2_PLACEMENT_3D ( 'NONE', #128909, #126953, #88283 ) ;
#112753=DIRECTION ( 'NONE',  ( 0.000000000000000000, -0.000000000000000000, 1.000000000000000000 ) ) ;
#112754=CARTESIAN_POINT ( 'NONE',  ( 13.74999999999989875, 2.500000000000000000, 1.472243186433545459 ) ) ;
#112755=DIRECTION ( 'NONE',  ( -0.000000000000000000, 1.000000000000000000, -0.000000000000000000 ) ) ;
#112756=LINE ( 'NONE', #2143, #30846 ) ;
#112757=ORIENTED_EDGE ( 'NONE', *, *, #51665, .F. ) ;
#112758=VECTOR ( 'NONE', #82032, 1000.000000000000000 ) ;
#112759=CONICAL_SURFACE ( 'NONE', #52118, 0.09999999999999982514, 0.003490658503988666988 ) ;
#112760=CARTESIAN_POINT ( 'NONE',  ( 13.94999999999989626, 12.50000000000000000, 2.446380397790835826 ) ) ;
#112761=ORIENTED_EDGE ( 'NONE', *, *, #99411, .F. ) ;
#112762=VECTOR ( 'NONE', #78635, 1000.000000000000000 ) ;
#112763=EDGE_LOOP ( 'NONE', ( #28853, #78456 ) ) ;
#112764=ORIENTED_EDGE ( 'NONE', *, *, #119597, .F. ) ;
#112765=DIRECTION ( 'NONE',  ( -0.000000000000000000, 1.000000000000000000, -0.000000000000000000 ) ) ;
#112766=ORIENTED_EDGE ( 'NONE', *, *, #18952, .T. ) ;
#112767=EDGE_LOOP ( 'NONE', ( #6297, #28633, #8022, #96027 ) ) ;
#112768=ORIENTED_EDGE ( 'NONE', *, *, #126486, .T. ) ;
#112769=AXIS2_PLACEMENT_3D ( 'NONE', #38151, #97704, #37519 ) ;
#112770=CARTESIAN_POINT ( 'NONE',  ( -5.200000000000022382, 2.500000000000000000, 4.776537180435972196 ) ) ;
#112771=CONICAL_SURFACE ( 'NONE', #83525, 0.09999999999999982514, 0.003490658503988666988 ) ;
#112772=ADVANCED_FACE ( 'NONE', ( #98796 ), #51020, .T. ) ;
#112773=DIRECTION ( 'NONE',  ( 0.000000000000000000, -0.9999939076577903929, 0.003490651415223739937 ) ) ;
#112774=DIRECTION ( 'NONE',  ( 0.000000000000000000, 0.000000000000000000, -1.000000000000000000 ) ) ;
#112775=CIRCLE ( 'NONE', #56312, 0.06509327318403745899 ) ;
#112776=LINE ( 'NONE', #34873, #94457 ) ;
#112777=LINE ( 'NONE', #35508, #82249 ) ;
#112778=DIRECTION ( 'NONE',  ( 0.000000000000000000, -0.9999939076577903929, 0.003490651415223739937 ) ) ;
#112779=EDGE_CURVE ( 'NONE', #21147, #92182, #70575, .T. ) ;
#112780=EDGE_LOOP ( 'NONE', ( #107964, #78214 ) ) ;
#112781=DIRECTION ( 'NONE',  ( 0.000000000000000000, 0.000000000000000000, 1.000000000000000000 ) ) ;
#112782=VERTEX_POINT ( 'NONE', #119728 ) ;
#112783=CARTESIAN_POINT ( 'NONE',  ( 5.799999999999931433, 2.500000000000000000, 4.230127018922196669 ) ) ;
#112784=AXIS2_PLACEMENT_3D ( 'NONE', #28608, #128759, #27954 ) ;
#112785=VERTEX_POINT ( 'NONE', #30094 ) ;
#112786=CARTESIAN_POINT ( 'NONE',  ( -6.450000000000016165, 12.50000000000000000, 2.511473670974873507 ) ) ;
#112787=ADVANCED_FACE ( 'NONE', ( #100729 ), #109931, .T. ) ;
#112788=EDGE_CURVE ( 'NONE', #7747, #80502, #18335, .T. ) ;
#112789=ORIENTED_EDGE ( 'NONE', *, *, #51523, .T. ) ;
#112791=EDGE_CURVE ( 'NONE', #7975, #112855, #1257, .T. ) ;
#112792=FACE_OUTER_BOUND ( 'NONE', #95615, .T. ) ;
#112793=ORIENTED_EDGE ( 'NONE', *, *, #72879, .F. ) ;
#112794=ORIENTED_EDGE ( 'NONE', *, *, #81648, .T. ) ;
#112795=CARTESIAN_POINT ( 'NONE',  ( 15.19999999999989093, 2.500000000000000000, 0.4464101615137735513 ) ) ;
#112796=DIRECTION ( 'NONE',  ( 0.000000000000000000, 0.000000000000000000, 1.000000000000000000 ) ) ;
#112797=EDGE_CURVE ( 'NONE', #38962, #118209, #63402, .T. ) ;
#112798=DIRECTION ( 'NONE',  ( -0.000000000000000000, 1.000000000000000000, -0.000000000000000000 ) ) ;
#112799=DIRECTION ( 'NONE',  ( 0.000000000000000000, -0.9999939076577903929, 0.003490651415223739937 ) ) ;
#112800=CIRCLE ( 'NONE', #8224, 0.06509327318403745899 ) ;
#112801=DIRECTION ( 'NONE',  ( 0.000000000000000000, 0.000000000000000000, 1.000000000000000000 ) ) ;
#112802=EDGE_LOOP ( 'NONE', ( #13975, #45873 ) ) ;
#112803=CARTESIAN_POINT ( 'NONE',  ( -4.150000000000028777, 12.50000000000000000, -5.802370205355749988 ) ) ;
#112804=AXIS2_PLACEMENT_3D ( 'NONE', #66369, #106298, #56542 ) ;
#112805=ORIENTED_EDGE ( 'NONE', *, *, #115264, .T. ) ;
#112806=DIRECTION ( 'NONE',  ( 0.000000000000000000, 0.000000000000000000, 1.000000000000000000 ) ) ;
#112807=CARTESIAN_POINT ( 'NONE',  ( 9.199999999999919353, 2.500000000000000000, -2.276824562219559311E-15 ) ) ;
#112808=CIRCLE ( 'NONE', #66727, 0.1000000000000002554 ) ;
#112809=CIRCLE ( 'NONE', #89809, 0.06509327318403745899 ) ;
#112810=AXIS2_PLACEMENT_3D ( 'NONE', #124626, #12718, #4829 ) ;
#112812=DIRECTION ( 'NONE',  ( 0.000000000000000000, 1.000000000000000000, 0.000000000000000000 ) ) ;
#112813=FACE_OUTER_BOUND ( 'NONE', #120868, .T. ) ;
#112814=CARTESIAN_POINT ( 'NONE',  ( 9.999999999999916511, 2.500000000000000000, -0.6928203230275541413 ) ) ;
#112815=DIRECTION ( 'NONE',  ( 0.000000000000000000, 0.000000000000000000, 1.000000000000000000 ) ) ;
#112816=VERTEX_POINT ( 'NONE', #12356 ) ;
#112817=CIRCLE ( 'NONE', #18718, 0.06509327318403741736 ) ;
#112818=VECTOR ( 'NONE', #112671, 1000.000000000000000 ) ;
#112819=FACE_OUTER_BOUND ( 'NONE', #37462, .T. ) ;
#112820=ADVANCED_FACE ( 'NONE', ( #64680 ), #51807, .T. ) ;
#112821=CARTESIAN_POINT ( 'NONE',  ( -2.900000000000029221, 2.500000000000000000, -0.7928203230275542301 ) ) ;
#112822=CARTESIAN_POINT ( 'NONE',  ( -2.700000000000030820, 12.50000000000000000, 0.3464101615137735735 ) ) ;
#112823=ORIENTED_EDGE ( 'NONE', *, *, #111622, .T. ) ;
#112825=DIRECTION ( 'NONE',  ( 0.000000000000000000, 0.000000000000000000, 1.000000000000000000 ) ) ;
#112826=ORIENTED_EDGE ( 'NONE', *, *, #101609, .T. ) ;
#112827=EDGE_LOOP ( 'NONE', ( #129507, #22385 ) ) ;
#112828=DIRECTION ( 'NONE',  ( -0.000000000000000000, 1.000000000000000000, -0.000000000000000000 ) ) ;
#112829=EDGE_CURVE ( 'NONE', #63919, #108022, #62766, .T. ) ;
#112830=EDGE_LOOP ( 'NONE', ( #91249, #4084, #51755, #21507 ) ) ;
#112831=CARTESIAN_POINT ( 'NONE',  ( 20.37025966759390272, -0.6621301594381256983, -4.188616773932661630 ) ) ;
#112832=DIRECTION ( 'NONE',  ( 0.000000000000000000, -0.000000000000000000, 1.000000000000000000 ) ) ;
#112833=EDGE_CURVE ( 'NONE', #47021, #10500, #3768, .T. ) ;
#112834=DIRECTION ( 'NONE',  ( -4.274815082592931898E-19, -0.9999939076577903929, -0.003490651415223739937 ) ) ;
#112835=ADVANCED_FACE ( 'NONE', ( #24771 ), #35085, .T. ) ;
#112836=ORIENTED_EDGE ( 'NONE', *, *, #12052, .F. ) ;
#112837=LINE ( 'NONE', #93837, #69668 ) ;
#112838=CIRCLE ( 'NONE', #14521, 0.06509327318403745899 ) ;
#112839=EDGE_CURVE ( 'NONE', #128265, #28777, #122907, .T. ) ;
#112840=DIRECTION ( 'NONE',  ( 0.000000000000000000, 0.000000000000000000, 1.000000000000000000 ) ) ;
#112841=ORIENTED_EDGE ( 'NONE', *, *, #81343, .T. ) ;
#112842=AXIS2_PLACEMENT_3D ( 'NONE', #20691, #40338, #71073 ) ;
#112843=VECTOR ( 'NONE', #85212, 1000.000000000000000 ) ;
#112844=EDGE_CURVE ( 'NONE', #42007, #70518, #55983, .T. ) ;
#112845=EDGE_CURVE ( 'NONE', #40379, #42733, #87289, .T. ) ;
#112846=VERTEX_POINT ( 'NONE', #122336 ) ;
#112847=ORIENTED_EDGE ( 'NONE', *, *, #16005, .F. ) ;
#112848=CARTESIAN_POINT ( 'NONE',  ( 0.8499999999999553468, 2.500000000000000000, 1.372243186433545370 ) ) ;
#112849=CARTESIAN_POINT ( 'NONE',  ( 6.649999999999927525, 12.50000000000000000, 2.165063509461097713 ) ) ;
#112850=DIRECTION ( 'NONE',  ( 0.000000000000000000, 0.000000000000000000, 1.000000000000000000 ) ) ;
#112851=ORIENTED_EDGE ( 'NONE', *, *, #3332, .T. ) ;
#112852=CIRCLE ( 'NONE', #41768, 0.1000000000000000056 ) ;
#112853=CARTESIAN_POINT ( 'NONE',  ( 4.999999999999935163, 12.50000000000000000, 0.6928203230275494784 ) ) ;
#112854=DIRECTION ( 'NONE',  ( 0.000000000000000000, 0.000000000000000000, 1.000000000000000000 ) ) ;
#112855=VERTEX_POINT ( 'NONE', #124258 ) ;
#112856=CONICAL_SURFACE ( 'NONE', #52308, 0.1000000000000002554, 0.003490658503988666988 ) ;
#112857=CARTESIAN_POINT ( 'NONE',  ( -0.8500000000000386136, 2.500000000000000000, 5.702370205355745014 ) ) ;
#112858=CARTESIAN_POINT ( 'NONE',  ( -10.65000000000000213, 2.500000000000000000, 6.048780366869520364 ) ) ;
#112860=DIRECTION ( 'NONE',  ( 0.000000000000000000, 0.000000000000000000, 1.000000000000000000 ) ) ;
#112861=DIRECTION ( 'NONE',  ( 0.000000000000000000, -0.9999939076577903929, 0.003490651415223739937 ) ) ;
#112862=CARTESIAN_POINT ( 'NONE',  ( 1.449999999999951328, 2.500000000000000000, -1.818653347947326138 ) ) ;
#112863=DIRECTION ( 'NONE',  ( -0.000000000000000000, 1.000000000000000000, -0.000000000000000000 ) ) ;
#112864=DIRECTION ( 'NONE',  ( 0.000000000000000000, 0.000000000000000000, 1.000000000000000000 ) ) ;
#112865=AXIS2_PLACEMENT_3D ( 'NONE', #4421, #104585, #24744 ) ;
#112866=ORIENTED_EDGE ( 'NONE', *, *, #24179, .F. ) ;
#112867=ORIENTED_EDGE ( 'NONE', *, *, #109950, .T. ) ;
#112868=ORIENTED_EDGE ( 'NONE', *, *, #66583, .F. ) ;
#112869=VERTEX_POINT ( 'NONE', #3204 ) ;
#112870=CIRCLE ( 'NONE', #58513, 0.06509327318403745899 ) ;
#112871=CARTESIAN_POINT ( 'NONE',  ( -1.900000000000034994, 12.50000000000000000, -0.4115034346978157509 ) ) ;
#112873=DIRECTION ( 'NONE',  ( -0.000000000000000000, 1.000000000000000000, -0.000000000000000000 ) ) ;
#112874=VERTEX_POINT ( 'NONE', #3831 ) ;
#112875=FACE_BOUND ( 'NONE', #36956, .T. ) ;
#112876=DIRECTION ( 'NONE',  ( 0.000000000000000000, 1.000000000000000000, 0.000000000000000000 ) ) ;
#112877=CARTESIAN_POINT ( 'NONE',  ( 10.64999999999990976, 12.50000000000000000, -6.776507416713039689 ) ) ;
#112878=CARTESIAN_POINT ( 'NONE',  ( 9.349999999999916156, 2.500000000000000000, 6.148780366869520009 ) ) ;
#112879=EDGE_CURVE ( 'NONE', #88979, #80302, #20505, .T. ) ;
#112880=DIRECTION ( 'NONE',  ( 0.000000000000000000, 0.000000000000000000, 1.000000000000000000 ) ) ;
#112881=DIRECTION ( 'NONE',  ( 0.000000000000000000, 0.000000000000000000, 1.000000000000000000 ) ) ;
#112883=( BOUNDED_CURVE ( )  B_SPLINE_CURVE ( 2, ( #67154, #99243, #58669 ),
 .UNSPECIFIED., .F., .F. ) 
 B_SPLINE_CURVE_WITH_KNOTS ( ( 3, 3 ),
 ( 0.000000000000000000, 0.01487798352592973813 ),
 .UNSPECIFIED. ) 
 CURVE ( )  GEOMETRIC_REPRESENTATION_ITEM ( )  RATIONAL_B_SPLINE_CURVE ( ( 0.8943752373141968803, 0.7762344340431478473, 1.000000000000000000 ) ) 
 REPRESENTATION_ITEM ( '' )  );
#112884=LINE ( 'NONE', #20643, #12051 ) ;
#112885=CARTESIAN_POINT ( 'NONE',  ( 0.8499999999999545697, 12.50000000000000000, 2.857883832488649301 ) ) ;
#112886=DIRECTION ( 'NONE',  ( 0.000000000000000000, 0.000000000000000000, 1.000000000000000000 ) ) ;
#112887=ORIENTED_EDGE ( 'NONE', *, *, #2807, .F. ) ;
#112888=ADVANCED_FACE ( 'NONE', ( #14283 ), #93764, .T. ) ;
#112889=EDGE_LOOP ( 'NONE', ( #33391, #35229 ) ) ;
#112890=ORIENTED_EDGE ( 'NONE', *, *, #91263, .F. ) ;
#112891=ORIENTED_EDGE ( 'NONE', *, *, #117518, .F. ) ;
#112892=ORIENTED_EDGE ( 'NONE', *, *, #105051, .F. ) ;
#112893=ORIENTED_EDGE ( 'NONE', *, *, #12470, .F. ) ;
#112894=CARTESIAN_POINT ( 'NONE',  ( 12.09999999999990550, 2.500000000000000000, 4.922947341949748257 ) ) ;
#112895=VECTOR ( 'NONE', #54301, 1000.000000000000000 ) ;
#112896=EDGE_LOOP ( 'NONE', ( #55245, #104171, #35376, #102044 ) ) ;
#112897=ORIENTED_EDGE ( 'NONE', *, *, #19225, .F. ) ;
#112898=AXIS2_PLACEMENT_3D ( 'NONE', #38276, #38946, #88655 ) ;
#112899=AXIS2_PLACEMENT_3D ( 'NONE', #39628, #70344, #108329 ) ;
#112900=CARTESIAN_POINT ( 'NONE',  ( 6.249999999999928946, 12.50000000000000000, 2.922977105672686982 ) ) ;
#112901=DIRECTION ( 'NONE',  ( 0.000000000000000000, 0.000000000000000000, 1.000000000000000000 ) ) ;
#112902=CARTESIAN_POINT ( 'NONE',  ( 12.49999999999990408, 2.500000000000000000, 4.922947341949748257 ) ) ;
#112903=EDGE_LOOP ( 'NONE', ( #51429, #73704 ) ) ;
#112904=DIRECTION ( 'NONE',  ( -0.000000000000000000, 1.000000000000000000, -0.000000000000000000 ) ) ;
#112905=CONICAL_SURFACE ( 'NONE', #23, 0.1000000000000000472, 0.003490658503988666988 ) ;
#112906=CIRCLE ( 'NONE', #39485, 0.1000000000000000472 ) ;
#112907=ORIENTED_EDGE ( 'NONE', *, *, #5060, .T. ) ;
#112908=ORIENTED_EDGE ( 'NONE', *, *, #116429, .F. ) ;
#112909=PLANE ( 'NONE',  #96989 ) ;
#112910=CARTESIAN_POINT ( 'NONE',  ( -12.04999999999999716, 2.500000000000000000, -2.165063509461097713 ) ) ;
#112911=ORIENTED_EDGE ( 'NONE', *, *, #100483, .F. ) ;
#112912=ORIENTED_EDGE ( 'NONE', *, *, #70288, .F. ) ;
#112913=CARTESIAN_POINT ( 'NONE',  ( 14.14999999999989200, 12.50000000000000000, -2.230156782645139391 ) ) ;
#112914=DIRECTION ( 'NONE',  ( -0.000000000000000000, -1.000000000000000000, -0.000000000000000000 ) ) ;
#112915=DIRECTION ( 'NONE',  ( -4.274815082592931898E-19, -0.9999939076577903929, -0.003490651415223739937 ) ) ;
#112916=CARTESIAN_POINT ( 'NONE',  ( -13.94999999999998863, 2.500000000000000000, 2.511473670974877503 ) ) ;
#112917=DIRECTION ( 'NONE',  ( 0.000000000000000000, -0.000000000000000000, 1.000000000000000000 ) ) ;
#112918=ORIENTED_EDGE ( 'NONE', *, *, #94990, .F. ) ;
#112919=CARTESIAN_POINT ( 'NONE',  ( 6.598553918464069135, -2.499999999999999556, 8.770211965307140645 ) ) ;
#112920=VECTOR ( 'NONE', #54951, 1000.000000000000000 ) ;
#112921=EDGE_CURVE ( 'NONE', #94312, #121167, #91504, .T. ) ;
#112922=AXIS2_PLACEMENT_3D ( 'NONE', #58495, #69572, #67632 ) ;
#112923=ORIENTED_EDGE ( 'NONE', *, *, #24906, .T. ) ;
#112924=CARTESIAN_POINT ( 'NONE',  ( 87.50000000000002842, 7.402262750143060899, -1.385127402881716430 ) ) ;
#112925=ORIENTED_EDGE ( 'NONE', *, *, #47669, .F. ) ;
#112926=CARTESIAN_POINT ( 'NONE',  ( 5.599999999999931255, 2.500000000000000000, 3.983716857408420076 ) ) ;
#112927=CARTESIAN_POINT ( 'NONE',  ( 13.94999999999989804, 2.500000000000000000, 1.718653347947321386 ) ) ;
#112928=DIRECTION ( 'NONE',  ( 0.000000000000000000, 0.000000000000000000, 1.000000000000000000 ) ) ;
#112929=ADVANCED_FACE ( 'NONE', ( #107175 ), #124952, .T. ) ;
#112930=CARTESIAN_POINT ( 'NONE',  ( -12.49999999999999467, 2.500000000000000000, -3.537306695894647302 ) ) ;
#112931=EDGE_CURVE ( 'NONE', #10496, #46288, #26696, .T. ) ;
#112932=EDGE_LOOP ( 'NONE', ( #103900, #124693 ) ) ;
#112933=CIRCLE ( 'NONE', #2103, 0.06509327318403745899 ) ;
#112934=CARTESIAN_POINT ( 'NONE',  ( -10.85000000000000142, 2.500000000000000000, -2.265063509461097802 ) ) ;
#112935=EDGE_CURVE ( 'NONE', #13848, #77485, #5741, .T. ) ;
#112936=CARTESIAN_POINT ( 'NONE',  ( -8.150000000000012790, 12.50000000000000000, -1.818653347947326138 ) ) ;
#112937=EDGE_LOOP ( 'NONE', ( #85144, #45960, #46101, #114274 ) ) ;
#112938=EDGE_CURVE ( 'NONE', #77431, #9926, #105902, .T. ) ;
#112939=ORIENTED_EDGE ( 'NONE', *, *, #112921, .F. ) ;
#112940=ORIENTED_EDGE ( 'NONE', *, *, #16974, .T. ) ;
#112941=DIRECTION ( 'NONE',  ( -0.000000000000000000, 1.000000000000000000, -0.000000000000000000 ) ) ;
#112942=DIRECTION ( 'NONE',  ( 0.000000000000000000, 0.000000000000000000, -1.000000000000000000 ) ) ;
#112943=EDGE_CURVE ( 'NONE', #21757, #125307, #26750, .T. ) ;
#112945=CIRCLE ( 'NONE', #62780, 0.1000000000000002554 ) ;
#112946=FACE_OUTER_BOUND ( 'NONE', #68623, .T. ) ;
#112947=DIRECTION ( 'NONE',  ( 0.000000000000000000, 0.000000000000000000, 1.000000000000000000 ) ) ;
#112948=AXIS2_PLACEMENT_3D ( 'NONE', #45842, #56288, #66113 ) ;
#112949=AXIS2_PLACEMENT_3D ( 'NONE', #36543, #33954, #3838 ) ;
#112950=CARTESIAN_POINT ( 'NONE',  ( -12.89999999999999325, 12.50000000000000000, 0.6277270498435161272 ) ) ;
#112952=ORIENTED_EDGE ( 'NONE', *, *, #31132, .T. ) ;
#112953=DIRECTION ( 'NONE',  ( 0.000000000000000000, 0.000000000000000000, 1.000000000000000000 ) ) ;
#112954=ORIENTED_EDGE ( 'NONE', *, *, #5844, .T. ) ;
#112955=CONICAL_SURFACE ( 'NONE', #102494, 0.1000000000000002554, 0.003490658503988666988 ) ;
#112956=DIRECTION ( 'NONE',  ( 0.000000000000000000, -0.9999939076577903929, 0.003490651415223739937 ) ) ;
#112957=DIRECTION ( 'NONE',  ( -0.000000000000000000, -1.000000000000000000, -0.000000000000000000 ) ) ;
#112958=DIRECTION ( 'NONE',  ( 0.000000000000000000, -0.9999939076577903929, 0.003490651415223739937 ) ) ;
#112959=CARTESIAN_POINT ( 'NONE',  ( -0.6000000000000388356, 2.500000000000000000, 4.676537180435972552 ) ) ;
#112960=ORIENTED_EDGE ( 'NONE', *, *, #121972, .T. ) ;
#112961=CARTESIAN_POINT ( 'NONE',  ( -10.45000000000000462, 2.500000000000000000, -6.495190528383298911 ) ) ;
#112962=DIRECTION ( 'NONE',  ( 0.000000000000000000, 0.000000000000000000, -1.000000000000000000 ) ) ;
#112963=CARTESIAN_POINT ( 'NONE',  ( -11.64999999999999680, 2.500000000000000000, 6.495190528383297135 ) ) ;
#112964=ORIENTED_EDGE ( 'NONE', *, *, #37156, .T. ) ;
#112965=ORIENTED_EDGE ( 'NONE', *, *, #6045, .T. ) ;
#112966=DIRECTION ( 'NONE',  ( 0.000000000000000000, 0.000000000000000000, -1.000000000000000000 ) ) ;
#112967=ORIENTED_EDGE ( 'NONE', *, *, #89485, .T. ) ;
#112968=ORIENTED_EDGE ( 'NONE', *, *, #16112, .F. ) ;
#112969=CARTESIAN_POINT ( 'NONE',  ( -7.900000000000014566, 2.500000000000000000, -5.022947341949754119 ) ) ;
#112970=VECTOR ( 'NONE', #91989, 1000.000000000000000 ) ;
#112971=EDGE_CURVE ( 'NONE', #84933, #17899, #24606, .T. ) ;
#112972=ADVANCED_FACE ( 'NONE', ( #107831 ), #110371, .T. ) ;
#112973=VECTOR ( 'NONE', #84242, 1000.000000000000000 ) ;
#112974=VERTEX_POINT ( 'NONE', #15571 ) ;
#112975=CARTESIAN_POINT ( 'NONE',  ( -0.6000000000000383915, 12.50000000000000000, -4.741630453620015118 ) ) ;
#112976=CARTESIAN_POINT ( 'NONE',  ( 8.299999999999922551, 2.500000000000000000, -0.1000000000000023925 ) ) ;
#112977=EDGE_CURVE ( 'NONE', #84112, #2963, #1605, .T. ) ;
#112978=DIRECTION ( 'NONE',  ( 0.000000000000000000, 1.000000000000000000, 0.000000000000000000 ) ) ;
#112979=VERTEX_POINT ( 'NONE', #27982 ) ;
#112980=CONICAL_SURFACE ( 'NONE', #35632, 0.1000000000000002554, 0.003490658503988666988 ) ;
#112981=DIRECTION ( 'NONE',  ( 0.000000000000000000, -0.000000000000000000, 1.000000000000000000 ) ) ;
#112982=CARTESIAN_POINT ( 'NONE',  ( 10.84999999999991260, 12.50000000000000000, -2.792790559304616504 ) ) ;
#112983=VERTEX_POINT ( 'NONE', #47628 ) ;
#112984=EDGE_CURVE ( 'NONE', #15707, #125017, #45545, .T. ) ;
#112985=CARTESIAN_POINT ( 'NONE',  ( 10.19999999999991225, 12.50000000000000000, -4.676537180435978769 ) ) ;
#112986=ADVANCED_FACE ( 'NONE', ( #116352 ), #16256, .T. ) ;
#112988=ADVANCED_FACE ( 'NONE', ( #58097 ), #12075, .T. ) ;
#112989=VERTEX_POINT ( 'NONE', #21887 ) ;
#112990=ADVANCED_FACE ( 'NONE', ( #68541 ), #62039, .T. ) ;
#112991=EDGE_CURVE ( 'NONE', #15146, #97073, #68509, .T. ) ;
#112992=EDGE_LOOP ( 'NONE', ( #17510, #18554 ) ) ;
#112993=ORIENTED_EDGE ( 'NONE', *, *, #76470, .T. ) ;
#112994=EDGE_LOOP ( 'NONE', ( #81440, #80602, #53462, #37801 ) ) ;
#112995=LINE ( 'NONE', #124748, #37910 ) ;
#112996=CARTESIAN_POINT ( 'NONE',  ( -10.85000000000000142, 2.500000000000000000, -5.802370205355746435 ) ) ;
#112997=DIRECTION ( 'NONE',  ( -4.274815082592931898E-19, -0.9999939076577903929, -0.003490651415223739937 ) ) ;
#112998=FACE_BOUND ( 'NONE', #47254, .T. ) ;
#112999=EDGE_LOOP ( 'NONE', ( #22252, #57821 ) ) ;
#113001=EDGE_CURVE ( 'NONE', #117215, #129515, #21216, .T. ) ;
#113002=CARTESIAN_POINT ( 'NONE',  ( 6.049999999999934097, 2.500000000000000000, 6.148780366869520897 ) ) ;
#113003=CARTESIAN_POINT ( 'NONE',  ( -14.34999999999998543, 2.500000000000000000, -2.611473670974875372 ) ) ;
#113004=CARTESIAN_POINT ( 'NONE',  ( -2.700000000000031264, 2.500000000000000000, 4.676537180435972552 ) ) ;
#113005=CARTESIAN_POINT ( 'NONE',  ( -10.20000000000000462, 2.500000000000000000, 0.4464101615137735513 ) ) ;
#113006=DIRECTION ( 'NONE',  ( 0.000000000000000000, 1.000000000000000000, 0.000000000000000000 ) ) ;
#113007=CONICAL_SURFACE ( 'NONE', #62841, 0.1000000000000000472, 0.003490658503988666988 ) ;
#113008=CIRCLE ( 'NONE', #23130, 0.06509327318403745899 ) ;
#113009=CARTESIAN_POINT ( 'NONE',  ( 4.599999999999938360, 12.50000000000000000, -0.7579135962115916003 ) ) ;
#113010=ORIENTED_EDGE ( 'NONE', *, *, #19553, .F. ) ;
#113011=VERTEX_POINT ( 'NONE', #11397 ) ;
#113012=EDGE_LOOP ( 'NONE', ( #34589, #107063, #115088, #63118 ) ) ;
#113013=VERTEX_POINT ( 'NONE', #101726 ) ;
#113014=ORIENTED_EDGE ( 'NONE', *, *, #119280, .F. ) ;
#113015=DIRECTION ( 'NONE',  ( 0.000000000000000000, 1.000000000000000000, 0.000000000000000000 ) ) ;
#113016=DIRECTION ( 'NONE',  ( 0.000000000000000000, 1.000000000000000000, 0.000000000000000000 ) ) ;
#113017=ORIENTED_EDGE ( 'NONE', *, *, #36480, .F. ) ;
#113018=FACE_BOUND ( 'NONE', #123128, .T. ) ;
#113019=AXIS2_PLACEMENT_3D ( 'NONE', #118936, #105899, #46325 ) ;
#113020=DIRECTION ( 'NONE',  ( 0.000000000000000000, -0.9999939076577903929, 0.003490651415223739937 ) ) ;
#113021=VERTEX_POINT ( 'NONE', #41534 ) ;
#113022=LINE ( 'NONE', #102552, #57878 ) ;
#113023=DIRECTION ( 'NONE',  ( 0.000000000000000000, 0.000000000000000000, 1.000000000000000000 ) ) ;
#113024=DIRECTION ( 'NONE',  ( 0.000000000000000000, 0.000000000000000000, 1.000000000000000000 ) ) ;
#113025=ORIENTED_EDGE ( 'NONE', *, *, #102176, .T. ) ;
#113026=DIRECTION ( 'NONE',  ( -0.000000000000000000, 1.000000000000000000, -0.000000000000000000 ) ) ;
#113027=AXIS2_PLACEMENT_3D ( 'NONE', #119723, #129583, #80474 ) ;
#113028=EDGE_LOOP ( 'NONE', ( #2962, #42412, #32107, #54209 ) ) ;
#113029=CIRCLE ( 'NONE', #145, 0.06509327318403745899 ) ;
#113030=EDGE_CURVE ( 'NONE', #78724, #4520, #118687, .T. ) ;
#113031=ORIENTED_EDGE ( 'NONE', *, *, #109842, .F. ) ;
#113032=ORIENTED_EDGE ( 'NONE', *, *, #69248, .T. ) ;
#113033=CARTESIAN_POINT ( 'NONE',  ( -9.350000000000006750, 2.500000000000000000, -2.511473670974877948 ) ) ;
#113034=DIRECTION ( 'NONE',  ( 0.000000000000000000, 1.000000000000000000, 0.000000000000000000 ) ) ;
#113035=DIRECTION ( 'NONE',  ( -0.000000000000000000, 1.000000000000000000, -0.000000000000000000 ) ) ;
#113036=VERTEX_POINT ( 'NONE', #91899 ) ;
#113037=DIRECTION ( 'NONE',  ( 0.000000000000000000, 0.000000000000000000, -1.000000000000000000 ) ) ;
#113038=CONICAL_SURFACE ( 'NONE', #127708, 0.1000000000000000472, 0.003490658503988666988 ) ;
#113039=DIRECTION ( 'NONE',  ( 0.000000000000000000, 0.000000000000000000, -1.000000000000000000 ) ) ;
#113040=CARTESIAN_POINT ( 'NONE',  ( 9.999999999999916511, 2.500000000000000000, -0.7928203230275542301 ) ) ;
#113041=VECTOR ( 'NONE', #16074, 1000.000000000000000 ) ;
#113043=ORIENTED_EDGE ( 'NONE', *, *, #14966, .T. ) ;
#113044=CARTESIAN_POINT ( 'NONE',  ( 13.94999999999989448, 2.500000000000000000, -2.511473670974877948 ) ) ;
#113045=ORIENTED_EDGE ( 'NONE', *, *, #69631, .T. ) ;
#113047=ORIENTED_EDGE ( 'NONE', *, *, #94141, .F. ) ;
#113048=EDGE_LOOP ( 'NONE', ( #73070, #16643, #107269, #114369 ) ) ;
#113049=DIRECTION ( 'NONE',  ( 0.000000000000000000, 0.000000000000000000, 1.000000000000000000 ) ) ;
#113051=DIRECTION ( 'NONE',  ( 0.000000000000000000, 0.000000000000000000, 1.000000000000000000 ) ) ;
#113052=DIRECTION ( 'NONE',  ( -0.000000000000000000, -1.000000000000000000, -0.000000000000000000 ) ) ;
#113053=DIRECTION ( 'NONE',  ( 0.000000000000000000, 0.000000000000000000, 1.000000000000000000 ) ) ;
#113054=ORIENTED_EDGE ( 'NONE', *, *, #7799, .T. ) ;
#113055=ORIENTED_EDGE ( 'NONE', *, *, #54879, .F. ) ;
#113056=DIRECTION ( 'NONE',  ( 0.000000000000000000, 0.000000000000000000, -1.000000000000000000 ) ) ;
#113057=CARTESIAN_POINT ( 'NONE',  ( 3.149999999999946176, 2.500000000000000000, -2.411473670974877859 ) ) ;
#113058=AXIS2_PLACEMENT_3D ( 'NONE', #70110, #128406, #119844 ) ;
#113059=DIRECTION ( 'NONE',  ( -0.000000000000000000, -1.000000000000000000, -0.000000000000000000 ) ) ;
#113061=VERTEX_POINT ( 'NONE', #42156 ) ;
#113062=CIRCLE ( 'NONE', #58697, 0.09999999999999999167 ) ;
#113063=DIRECTION ( 'NONE',  ( 0.000000000000000000, 1.000000000000000000, 0.000000000000000000 ) ) ;
#113064=VERTEX_POINT ( 'NONE', #82741 ) ;
#113065=FACE_OUTER_BOUND ( 'NONE', #32363, .T. ) ;
#113066=PLANE ( 'NONE',  #39438 ) ;
#113067=EDGE_CURVE ( 'NONE', #31853, #31716, #79003, .T. ) ;
#113068=CONICAL_SURFACE ( 'NONE', #123438, 0.1000000000000000472, 0.003490658503988666988 ) ;
#113069=DIRECTION ( 'NONE',  ( 0.000000000000000000, 0.000000000000000000, 1.000000000000000000 ) ) ;
#113070=EDGE_LOOP ( 'NONE', ( #92074, #21817 ) ) ;
#113071=DIRECTION ( 'NONE',  ( 0.000000000000000000, 0.000000000000000000, 1.000000000000000000 ) ) ;
#113072=FACE_OUTER_BOUND ( 'NONE', #68689, .T. ) ;
#113073=CARTESIAN_POINT ( 'NONE',  ( -6.850000000000013856, 2.500000000000000000, 6.841600689897072485 ) ) ;
#113074=CARTESIAN_POINT ( 'NONE',  ( 9.149999999999916866, 2.500000000000000000, -2.857883832488653741 ) ) ;
#113075=AXIS2_PLACEMENT_3D ( 'NONE', #101162, #33085, #41613 ) ;
#113076=EDGE_CURVE ( 'NONE', #56218, #71451, #95764, .T. ) ;
#113078=EDGE_CURVE ( 'NONE', #62072, #94563, #37561, .T. ) ;
#113079=VERTEX_POINT ( 'NONE', #123921 ) ;
#113080=CARTESIAN_POINT ( 'NONE',  ( -2.300000000000032685, 2.500000000000000000, -4.676537180435978769 ) ) ;
#113081=CARTESIAN_POINT ( 'NONE',  ( 21.24754738303277790, -0.7337760880902381988, 4.182111650399363612 ) ) ;
#113082=ADVANCED_FACE ( 'NONE', ( #25086 ), #73530, .T. ) ;
#113083=EDGE_LOOP ( 'NONE', ( #99116, #67312, #1279, #26961 ) ) ;
#113084=EDGE_CURVE ( 'NONE', #120997, #94406, #114892, .T. ) ;
#113085=ORIENTED_EDGE ( 'NONE', *, *, #8951, .F. ) ;
#113086=EDGE_CURVE ( 'NONE', #85023, #97932, #123289, .T. ) ;
#113088=CARTESIAN_POINT ( 'NONE',  ( 11.44999999999990692, 2.500000000000000000, -6.841600689897078702 ) ) ;
#113089=EDGE_CURVE ( 'NONE', #35141, #45163, #52130, .T. ) ;
#113090=ADVANCED_FACE ( 'NONE', ( #63733 ), #125287, .T. ) ;
#113091=DIRECTION ( 'NONE',  ( 0.000000000000000000, 0.000000000000000000, -1.000000000000000000 ) ) ;
#113092=DIRECTION ( 'NONE',  ( 0.000000000000000000, 1.000000000000000000, 0.000000000000000000 ) ) ;
#113093=CARTESIAN_POINT ( 'NONE',  ( -3.350000000000028955, 2.500000000000000000, 5.902370205355745192 ) ) ;
#113094=CONICAL_SURFACE ( 'NONE', #14864, 0.1000000000000002554, 0.003490658503988666988 ) ;
#113095=DIRECTION ( 'NONE',  ( 0.000000000000000000, 1.000000000000000000, 0.000000000000000000 ) ) ;
#113096=DIRECTION ( 'NONE',  ( 0.000000000000000000, 1.000000000000000000, 0.000000000000000000 ) ) ;
#113097=DIRECTION ( 'NONE',  ( -4.274815082592931898E-19, -0.9999939076577903929, -0.003490651415223739937 ) ) ;
#113098=DIRECTION ( 'NONE',  ( 0.000000000000000000, -0.000000000000000000, 1.000000000000000000 ) ) ;
#113099=EDGE_CURVE ( 'NONE', #72352, #114066, #10355, .T. ) ;
#113100=DIRECTION ( 'NONE',  ( -0.000000000000000000, -1.000000000000000000, -0.000000000000000000 ) ) ;
#113101=AXIS2_PLACEMENT_3D ( 'NONE', #68673, #18917, #9109 ) ;
#113102=ORIENTED_EDGE ( 'NONE', *, *, #117054, .T. ) ;
#113103=ADVANCED_FACE ( 'NONE', ( #85292 ), #43460, .T. ) ;
#113104=EDGE_LOOP ( 'NONE', ( #32913, #128538 ) ) ;
#113105=ORIENTED_EDGE ( 'NONE', *, *, #86039, .T. ) ;
#113106=ORIENTED_EDGE ( 'NONE', *, *, #35834, .F. ) ;
#113107=CARTESIAN_POINT ( 'NONE',  ( -9.800000000000006040, 12.50000000000000000, 0.3464101615137735735 ) ) ;
#113108=PLANE ( 'NONE',  #16505 ) ;
#113109=AXIS2_PLACEMENT_3D ( 'NONE', #126988, #104741, #105414 ) ;
#113110=CIRCLE ( 'NONE', #27420, 0.1000000000000000472 ) ;
#113111=ORIENTED_EDGE ( 'NONE', *, *, #82820, .F. ) ;
#113112=FACE_OUTER_BOUND ( 'NONE', #71999, .T. ) ;
#113113=DIRECTION ( 'NONE',  ( 0.000000000000000000, 0.000000000000000000, -1.000000000000000000 ) ) ;
#113115=VERTEX_POINT ( 'NONE', #93832 ) ;
#113116=CARTESIAN_POINT ( 'NONE',  ( -0.4500000000000402012, 12.50000000000000000, 2.230156782645134950 ) ) ;
#113117=CARTESIAN_POINT ( 'NONE',  ( -4.350000000000023626, 12.50000000000000000, -1.818653347947325916 ) ) ;
#113118=AXIS2_PLACEMENT_3D ( 'NONE', #116343, #56761, #86229 ) ;
#113119=VERTEX_POINT ( 'NONE', #75469 ) ;
#113120=CIRCLE ( 'NONE', #73406, 0.06509327318403743123 ) ;
#113121=ORIENTED_EDGE ( 'NONE', *, *, #112833, .F. ) ;
#113122=ORIENTED_EDGE ( 'NONE', *, *, #39977, .T. ) ;
#113123=VERTEX_POINT ( 'NONE', #104914 ) ;
#113124=DIRECTION ( 'NONE',  ( 0.000000000000000000, 0.000000000000000000, -1.000000000000000000 ) ) ;
#113125=ADVANCED_FACE ( 'NONE', ( #26390 ), #8288, .T. ) ;
#113126=AXIS2_PLACEMENT_3D ( 'NONE', #101245, #112361, #122824 ) ;
#113127=DIRECTION ( 'NONE',  ( -0.000000000000000000, -1.000000000000000000, -0.000000000000000000 ) ) ;
#113128=DIRECTION ( 'NONE',  ( 0.000000000000000000, 1.000000000000000000, 0.000000000000000000 ) ) ;
#113129=EDGE_CURVE ( 'NONE', #71812, #126312, #100252, .T. ) ;
#113130=DIRECTION ( 'NONE',  ( -0.000000000000000000, -1.000000000000000000, -0.000000000000000000 ) ) ;
#113131=VERTEX_POINT ( 'NONE', #125854 ) ;
#113132=EDGE_CURVE ( 'NONE', #62174, #93106, #4135, .T. ) ;
#113133=CIRCLE ( 'NONE', #254, 0.1000000000000002554 ) ;
#113134=CIRCLE ( 'NONE', #63059, 0.1000000000000002554 ) ;
#113135=CARTESIAN_POINT ( 'NONE',  ( -9.400000000000009237, 2.500000000000000000, -4.676537180435974328 ) ) ;
#113136=ORIENTED_EDGE ( 'NONE', *, *, #85416, .T. ) ;
#113137=FACE_OUTER_BOUND ( 'NONE', #36157, .T. ) ;
#113138=CARTESIAN_POINT ( 'NONE',  ( 10.87377556668746514, -2.500000000000257128, -8.986829607522045293 ) ) ;
#113139=CARTESIAN_POINT ( 'NONE',  ( 1.649999999999951950, 2.500000000000000000, -5.902370205355750521 ) ) ;
#113140=DIRECTION ( 'NONE',  ( 0.000000000000000000, -0.000000000000000000, 1.000000000000000000 ) ) ;
#113141=EDGE_CURVE ( 'NONE', #59160, #87633, #65653, .T. ) ;
#113142=EDGE_CURVE ( 'NONE', #34124, #86025, #102311, .T. ) ;
#113143=ORIENTED_EDGE ( 'NONE', *, *, #60029, .T. ) ;
#113144=ADVANCED_FACE ( 'NONE', ( #114112 ), #108642, .T. ) ;
#113145=ORIENTED_EDGE ( 'NONE', *, *, #26127, .T. ) ;
#113146=VERTEX_POINT ( 'NONE', #24446 ) ;
#113147=CARTESIAN_POINT ( 'NONE',  ( -0.2000000000000347888, 2.500000000000000000, 0.2464101615137758439 ) ) ;
#113148=LINE ( 'NONE', #51671, #20553 ) ;
#113149=DIRECTION ( 'NONE',  ( -4.274815082592931898E-19, -0.9999939076577903929, -0.003490651415223739937 ) ) ;
#113150=FACE_BOUND ( 'NONE', #62567, .T. ) ;
#113151=DIRECTION ( 'NONE',  ( -0.000000000000000000, -1.000000000000000000, -0.000000000000000000 ) ) ;
#113152=CARTESIAN_POINT ( 'NONE',  ( -9.600000000000008527, 2.500000000000000000, -4.330127018922197202 ) ) ;
#113153=EDGE_CURVE ( 'NONE', #56350, #47664, #39633, .T. ) ;
#113154=DIRECTION ( 'NONE',  ( 0.000000000000000000, -0.9999939076577903929, 0.003490651415223739937 ) ) ;
#113155=CIRCLE ( 'NONE', #8584, 0.1000000000000002554 ) ;
#113156=VECTOR ( 'NONE', #9908, 1000.000000000000000 ) ;
#113157=DIRECTION ( 'NONE',  ( -0.000000000000000000, -1.000000000000000000, -0.000000000000000000 ) ) ;
#113158=CIRCLE ( 'NONE', #96417, 0.06509327318403745899 ) ;
#113160=CARTESIAN_POINT ( 'NONE',  ( -2.100000000000033396, 2.500000000000000000, 0.7928203230275495672 ) ) ;
#113161=ORIENTED_EDGE ( 'NONE', *, *, #37642, .F. ) ;
#113162=AXIS2_PLACEMENT_3D ( 'NONE', #117135, #117780, #47141 ) ;
#113163=DIRECTION ( 'NONE',  ( 0.000000000000000000, 0.000000000000000000, 1.000000000000000000 ) ) ;
#113164=CIRCLE ( 'NONE', #92227, 0.1000000000000002554 ) ;
#113165=VERTEX_POINT ( 'NONE', #46030 ) ;
#113166=ORIENTED_EDGE ( 'NONE', *, *, #16615, .T. ) ;
#113167=PLANE ( 'NONE',  #115532 ) ;
#113168=EDGE_CURVE ( 'NONE', #22620, #89608, #36211, .T. ) ;
#113169=FACE_BOUND ( 'NONE', #59394, .T. ) ;
#113170=CARTESIAN_POINT ( 'NONE',  ( 6.249999999999967137, 2.500000000000000000, -2.065063509461102065 ) ) ;
#113171=ORIENTED_EDGE ( 'NONE', *, *, #95137, .F. ) ;
#113172=CARTESIAN_POINT ( 'NONE',  ( 43.31214921617725366, 3.511364963952507967, 3.941696051818830870 ) ) ;
#113173=DIRECTION ( 'NONE',  ( -0.000000000000000000, 1.000000000000000000, -0.000000000000000000 ) ) ;
#113174=ORIENTED_EDGE ( 'NONE', *, *, #38009, .F. ) ;
#113175=DIRECTION ( 'NONE',  ( -4.274815082592931898E-19, -0.9999939076577903929, -0.003490651415223739937 ) ) ;
#113176=FACE_OUTER_BOUND ( 'NONE', #70953, .T. ) ;
#113177=EDGE_CURVE ( 'NONE', #109519, #125908, #116947, .T. ) ;
#113178=EDGE_LOOP ( 'NONE', ( #100462, #36932 ) ) ;
#113179=CARTESIAN_POINT ( 'NONE',  ( -6.650000000000019007, 2.500000000000000000, -5.702370205355749455 ) ) ;
#113180=FACE_OUTER_BOUND ( 'NONE', #41118, .T. ) ;
#113181=CIRCLE ( 'NONE', #106924, 0.06509327318403745899 ) ;
#113182=VERTEX_POINT ( 'NONE', #87217 ) ;
#113183=DIRECTION ( 'NONE',  ( -0.000000000000000000, 1.000000000000000000, -0.000000000000000000 ) ) ;
#113184=CARTESIAN_POINT ( 'NONE',  ( 2.499999999999945377, 2.500000000000000000, 5.022947341949748790 ) ) ;
#113186=EDGE_LOOP ( 'NONE', ( #81879, #123366 ) ) ;
#113187=ORIENTED_EDGE ( 'NONE', *, *, #3434, .F. ) ;
#113188=EDGE_CURVE ( 'NONE', #107957, #36304, #57119, .T. ) ;
#113190=CIRCLE ( 'NONE', #8723, 0.1000000000000000472 ) ;
#113191=ORIENTED_EDGE ( 'NONE', *, *, #7248, .F. ) ;
#113192=CARTESIAN_POINT ( 'NONE',  ( -3.750000000000027534, 12.50000000000000000, 2.857883832488649301 ) ) ;
#113193=CIRCLE ( 'NONE', #104774, 0.09999999999999982514 ) ;
#113194=CARTESIAN_POINT ( 'NONE',  ( 4.799999999999935874, 2.500000000000000000, 3.883716857408421319 ) ) ;
#113196=AXIS2_PLACEMENT_3D ( 'NONE', #57419, #56110, #128091 ) ;
#113197=DIRECTION ( 'NONE',  ( -4.274815082592931898E-19, -0.9999939076577903929, -0.003490651415223739937 ) ) ;
#113198=CARTESIAN_POINT ( 'NONE',  ( 9.999999999999948486, 12.50000000000000000, -4.395220292106239768 ) ) ;
#113199=FACE_OUTER_BOUND ( 'NONE', #68931, .T. ) ;
#113200=DIRECTION ( 'NONE',  ( -0.000000000000000000, 1.000000000000000000, -0.000000000000000000 ) ) ;
#113201=CARTESIAN_POINT ( 'NONE',  ( 11.64999999999990443, 2.500000000000000000, -5.802370205355749988 ) ) ;
#113202=CIRCLE ( 'NONE', #23319, 0.06509327318403741736 ) ;
#113203=VERTEX_POINT ( 'NONE', #47961 ) ;
#113204=PRODUCT_DEFINITION_FORMATION_WITH_SPECIFIED_SOURCE ( 'ANY', '', #33622, .NOT_KNOWN. ) ;
#113205=VECTOR ( 'NONE', #24463, 1000.000000000000000 ) ;
#113206=ORIENTED_EDGE ( 'NONE', *, *, #72882, .F. ) ;
#113207=CARTESIAN_POINT ( 'NONE',  ( 5.849999999999932143, 2.500000000000000000, 2.265063509461097357 ) ) ;
#113209=CIRCLE ( 'NONE', #54626, 0.1000000000000002554 ) ;
#113210=VERTEX_POINT ( 'NONE', #118618 ) ;
#113211=VERTEX_POINT ( 'NONE', #18484 ) ;
#113212=ORIENTED_EDGE ( 'NONE', *, *, #55940, .F. ) ;
#113213=DIRECTION ( 'NONE',  ( -0.000000000000000000, 1.000000000000000000, -0.000000000000000000 ) ) ;
#113214=CONICAL_SURFACE ( 'NONE', #125720, 0.09999999999999999167, 0.003490658503988666988 ) ;
#113215=CARTESIAN_POINT ( 'NONE',  ( 8.099999999999923261, 12.50000000000000000, -3.983716857408426293 ) ) ;
#113216=DIRECTION ( 'NONE',  ( 0.000000000000000000, 0.000000000000000000, -1.000000000000000000 ) ) ;
#113217=EDGE_CURVE ( 'NONE', #30225, #99143, #127441, .T. ) ;
#113219=CARTESIAN_POINT ( 'NONE',  ( -11.25000000000000178, 2.500000000000000000, -5.902370205355746968 ) ) ;
#113220=CIRCLE ( 'NONE', #123591, 0.06509327318403745899 ) ;
#113221=CIRCLE ( 'NONE', #52589, 0.06509327318403745899 ) ;
#113222=DIRECTION ( 'NONE',  ( 0.000000000000000000, 1.000000000000000000, 0.000000000000000000 ) ) ;
#113223=CARTESIAN_POINT ( 'NONE',  ( 14.79999999999989235, 12.50000000000000000, 0.3464101615137735735 ) ) ;
#113224=CARTESIAN_POINT ( 'NONE',  ( -4.400000000000025224, 12.50000000000000000, 3.983716857408420076 ) ) ;
#113225=CARTESIAN_POINT ( 'NONE',  ( -0.8500000000000382805, 2.500000000000000000, -7.088010851410853519 ) ) ;
#113226=CARTESIAN_POINT ( 'NONE',  ( 6.649999999999930189, 12.50000000000000000, -1.472243186433550122 ) ) ;
#113228=ORIENTED_EDGE ( 'NONE', *, *, #115816, .T. ) ;
#113229=LINE ( 'NONE', #22940, #42309 ) ;
#113230=ADVANCED_FACE ( 'NONE', ( #27641 ), #126518, .T. ) ;
#113231=VERTEX_POINT ( 'NONE', #69510 ) ;
#113232=EDGE_CURVE ( 'NONE', #69676, #20627, #12401, .T. ) ;
#113233=ORIENTED_EDGE ( 'NONE', *, *, #60773, .F. ) ;
#113234=ADVANCED_FACE ( 'NONE', ( #79357 ), #119257, .T. ) ;
#113235=CARTESIAN_POINT ( 'NONE',  ( 3.549999999999940314, 2.500000000000000000, 6.841600689897072485 ) ) ;
#113236=DIRECTION ( 'NONE',  ( 0.000000000000000000, -0.000000000000000000, 1.000000000000000000 ) ) ;
#113237=ADVANCED_FACE ( 'NONE', ( #66925 ), #119026, .T. ) ;
#113238=DIRECTION ( 'NONE',  ( 0.000000000000000000, 0.000000000000000000, -1.000000000000000000 ) ) ;
#113239=CARTESIAN_POINT ( 'NONE',  ( 9.399999999999915090, 12.50000000000000000, 4.676537180435972552 ) ) ;
#113240=CARTESIAN_POINT ( 'NONE',  ( -12.09999999999999609, 2.500000000000000000, -3.637306695894647390 ) ) ;
#113241=EDGE_CURVE ( 'NONE', #81692, #119348, #7367, .T. ) ;
#113242=CARTESIAN_POINT ( 'NONE',  ( 16.56576425165006583, -1.500000000000000666, 6.084390597445813675 ) ) ;
#113243=EDGE_CURVE ( 'NONE', #127958, #6155, #123238, .T. ) ;
#113244=AXIS2_PLACEMENT_3D ( 'NONE', #119117, #30759, #100744 ) ;
#113245=CARTESIAN_POINT ( 'NONE',  ( -11.05000000000000071, 12.50000000000000000, 6.841600689897072485 ) ) ;
#113246=EDGE_LOOP ( 'NONE', ( #99786, #47279, #39683, #42085 ) ) ;
#113248=CIRCLE ( 'NONE', #65117, 0.1000000000000002554 ) ;
#113249=CIRCLE ( 'NONE', #19138, 0.06509327318403745899 ) ;
#113250=ADVANCED_FACE ( 'NONE', ( #109447 ), #17839, .T. ) ;
#113251=CARTESIAN_POINT ( 'NONE',  ( -3.750000000000029310, 12.50000000000000000, -7.253104124594891289 ) ) ;
#113252=ADVANCED_FACE ( 'NONE', ( #116682 ), #79334, .T. ) ;
#113253=ORIENTED_EDGE ( 'NONE', *, *, #50072, .T. ) ;
#113254=CIRCLE ( 'NONE', #40104, 0.06509327318403745899 ) ;
#113255=ADVANCED_FACE ( 'NONE', ( #117969 ), #6138, .T. ) ;
#113256=ORIENTED_EDGE ( 'NONE', *, *, #112271, .T. ) ;
#113257=VECTOR ( 'NONE', #39679, 1000.000000000000000 ) ;
#113258=ORIENTED_EDGE ( 'NONE', *, *, #95510, .T. ) ;
#113259=CIRCLE ( 'NONE', #61027, 0.06509327318403745899 ) ;
#113260=AXIS2_PLACEMENT_3D ( 'NONE', #54521, #83363, #84642 ) ;
#113261=ORIENTED_EDGE ( 'NONE', *, *, #93326, .T. ) ;
#113262=EDGE_CURVE ( 'NONE', #109667, #65076, #68226, .T. ) ;
#113263=DIRECTION ( 'NONE',  ( -0.000000000000000000, -1.000000000000000000, -0.000000000000000000 ) ) ;
#113264=DIRECTION ( 'NONE',  ( 0.000000000000000000, 1.000000000000000000, 0.000000000000000000 ) ) ;
#113265=AXIS2_PLACEMENT_3D ( 'NONE', #75656, #103849, #124774 ) ;
#113266=DIRECTION ( 'NONE',  ( 0.000000000000000000, 1.000000000000000000, 0.000000000000000000 ) ) ;
#113267=FACE_OUTER_BOUND ( 'NONE', #48915, .T. ) ;
#113268=CARTESIAN_POINT ( 'NONE',  ( 13.29999999999990301, 2.500000000000000000, -4.330127018922201643 ) ) ;
#113269=ORIENTED_EDGE ( 'NONE', *, *, #23704, .T. ) ;
#113270=FACE_OUTER_BOUND ( 'NONE', #115049, .T. ) ;
#113271=CARTESIAN_POINT ( 'NONE',  ( -9.600000000000008527, 2.500000000000000000, -3.737306695894645259 ) ) ;
#113272=CARTESIAN_POINT ( 'NONE',  ( -9.200000000000006395, 12.50000000000000000, 4.330127018922196314 ) ) ;
#113273=CARTESIAN_POINT ( 'NONE',  ( 87.50000000000001421, 0.000000000000000000, 0.000000000000000000 ) ) ;
#113274=ORIENTED_EDGE ( 'NONE', *, *, #93469, .F. ) ;
#113275=ORIENTED_EDGE ( 'NONE', *, *, #124814, .T. ) ;
#113276=VERTEX_POINT ( 'NONE', #6698 ) ;
#113277=CARTESIAN_POINT ( 'NONE',  ( -15.19999999999998153, 12.50000000000000000, -0.4115034346978133639 ) ) ;
#113278=FACE_OUTER_BOUND ( 'NONE', #101365, .T. ) ;
#113279=AXIS2_PLACEMENT_3D ( 'NONE', #70458, #31823, #71753 ) ;
#113281=AXIS2_PLACEMENT_3D ( 'NONE', #34233, #31640, #74143 ) ;
#113282=ORIENTED_EDGE ( 'NONE', *, *, #54052, .T. ) ;
#113283=DIRECTION ( 'NONE',  ( 0.000000000000000000, 0.000000000000000000, -1.000000000000000000 ) ) ;
#113284=CARTESIAN_POINT ( 'NONE',  ( -6.450000000000014388, 2.500000000000000000, 1.818653347947321475 ) ) ;
#113286=CARTESIAN_POINT ( 'NONE',  ( -0.6500000000000389910, 12.50000000000000000, -6.148780366869526226 ) ) ;
#113287=AXIS2_PLACEMENT_3D ( 'NONE', #112985, #120237, #51503 ) ;
#113288=AXIS2_PLACEMENT_3D ( 'NONE', #82168, #102454, #12122 ) ;
#113289=EDGE_CURVE ( 'NONE', #118526, #18296, #22892, .T. ) ;
#113290=CIRCLE ( 'NONE', #17115, 0.1000000000000002554 ) ;
#113291=DIRECTION ( 'NONE',  ( 0.000000000000000000, 0.000000000000000000, 1.000000000000000000 ) ) ;
#113292=VECTOR ( 'NONE', #42285, 1000.000000000000000 ) ;
#113293=EDGE_CURVE ( 'NONE', #45906, #7993, #112775, .T. ) ;
#113295=EDGE_LOOP ( 'NONE', ( #74642, #15621, #100991, #8887 ) ) ;
#113296=CARTESIAN_POINT ( 'NONE',  ( 2.099999999999949463, 2.500000000000000000, -3.637306695894650055 ) ) ;
#113297=DIRECTION ( 'NONE',  ( 0.000000000000000000, 1.000000000000000000, 0.000000000000000000 ) ) ;
#113298=CARTESIAN_POINT ( 'NONE',  ( -5.450000000000023270, 2.500000000000000000, -2.065063509461102065 ) ) ;
#113299=DIRECTION ( 'NONE',  ( -0.000000000000000000, 1.000000000000000000, -0.000000000000000000 ) ) ;
#113300=AXIS2_PLACEMENT_3D ( 'NONE', #27813, #89321, #39606 ) ;
#113301=EDGE_CURVE ( 'NONE', #68377, #14536, #50517, .T. ) ;
#113302=VECTOR ( 'NONE', #119275, 1000.000000000000000 ) ;
#113303=CARTESIAN_POINT ( 'NONE',  ( 1.049999999999954969, 2.500000000000000000, -6.841600689897077814 ) ) ;
#113304=EDGE_LOOP ( 'NONE', ( #94816, #18419, #12083, #60200 ) ) ;
#113305=CIRCLE ( 'NONE', #94525, 0.09999999999999982514 ) ;
#113306=AXIS2_PLACEMENT_3D ( 'NONE', #27577, #46583, #86505 ) ;
#113307=AXIS2_PLACEMENT_3D ( 'NONE', #38708, #118517, #69412 ) ;
#113308=ORIENTED_EDGE ( 'NONE', *, *, #90962, .T. ) ;
#113309=DIRECTION ( 'NONE',  ( -0.000000000000000000, 1.000000000000000000, -0.000000000000000000 ) ) ;
#113310=DIRECTION ( 'NONE',  ( 0.000000000000000000, 1.000000000000000000, 0.000000000000000000 ) ) ;
#113311=DIRECTION ( 'NONE',  ( -0.000000000000000000, -1.000000000000000000, -0.000000000000000000 ) ) ;
#113312=AXIS2_PLACEMENT_3D ( 'NONE', #118473, #58286, #98192 ) ;
#113313=DIRECTION ( 'NONE',  ( 0.000000000000000000, 1.000000000000000000, 0.000000000000000000 ) ) ;
#113314=FACE_OUTER_BOUND ( 'NONE', #21831, .T. ) ;
#113315=ORIENTED_EDGE ( 'NONE', *, *, #30506, .T. ) ;
#113316=LINE ( 'NONE', #23012, #51097 ) ;
#113317=DIRECTION ( 'NONE',  ( 0.000000000000000000, -0.9999939076577903929, 0.003490651415223739937 ) ) ;
#113318=AXIS2_PLACEMENT_3D ( 'NONE', #36077, #14474, #116557 ) ;
#113319=ORIENTED_EDGE ( 'NONE', *, *, #61840, .F. ) ;
#113320=DIRECTION ( 'NONE',  ( 0.000000000000000000, 1.000000000000000000, 0.000000000000000000 ) ) ;
#113321=ORIENTED_EDGE ( 'NONE', *, *, #97279, .T. ) ;
#113322=DIRECTION ( 'NONE',  ( 0.000000000000000000, -0.9999939076577903929, 0.003490651415223739937 ) ) ;
#113323=EDGE_LOOP ( 'NONE', ( #116059, #49874, #24295, #111383 ) ) ;
#113324=DIRECTION ( 'NONE',  ( 0.000000000000000000, -0.000000000000000000, 1.000000000000000000 ) ) ;
#113326=ORIENTED_EDGE ( 'NONE', *, *, #12320, .T. ) ;
#113327=ORIENTED_EDGE ( 'NONE', *, *, #90165, .F. ) ;
#113329=DIRECTION ( 'NONE',  ( 0.000000000000000000, 0.000000000000000000, 1.000000000000000000 ) ) ;
#113330=CARTESIAN_POINT ( 'NONE',  ( 0.7999999999999553024, 12.50000000000000000, -4.330127018922201643 ) ) ;
#113332=CIRCLE ( 'NONE', #67337, 0.06509327318403745899 ) ;
#113333=LINE ( 'NONE', #102242, #11705 ) ;
#113334=CARTESIAN_POINT ( 'NONE',  ( 0.4499999999999573785, 2.500000000000000000, -6.395190528383301931 ) ) ;
#113336=FACE_OUTER_BOUND ( 'NONE', #28801, .T. ) ;
#113337=DIRECTION ( 'NONE',  ( 0.000000000000000000, 0.000000000000000000, -1.000000000000000000 ) ) ;
#113338=AXIS2_PLACEMENT_3D ( 'NONE', #123097, #22330, #84458 ) ;
#113339=ORIENTED_EDGE ( 'NONE', *, *, #69944, .F. ) ;
#113340=AXIS2_PLACEMENT_3D ( 'NONE', #108069, #129035, #79275 ) ;
#113341=ORIENTED_EDGE ( 'NONE', *, *, #29259, .T. ) ;
#113342=LINE ( 'NONE', #120593, #65338 ) ;
#113343=ORIENTED_EDGE ( 'NONE', *, *, #98150, .F. ) ;
#113344=DIRECTION ( 'NONE',  ( 0.000000000000000000, 1.000000000000000000, 0.000000000000000000 ) ) ;
#113345=DIRECTION ( 'NONE',  ( 0.000000000000000000, 0.000000000000000000, 1.000000000000000000 ) ) ;
#113346=EDGE_CURVE ( 'NONE', #61065, #42141, #52451, .T. ) ;
#113348=CIRCLE ( 'NONE', #125961, 0.06509327318403745899 ) ;
#113349=ORIENTED_EDGE ( 'NONE', *, *, #83826, .F. ) ;
#113350=ORIENTED_EDGE ( 'NONE', *, *, #34425, .T. ) ;
#113351=FACE_BOUND ( 'NONE', #112992, .T. ) ;
#113352=VERTEX_POINT ( 'NONE', #23006 ) ;
#113353=EDGE_CURVE ( 'NONE', #123245, #22096, #122497, .T. ) ;
#113354=CARTESIAN_POINT ( 'NONE',  ( 10.44999999999991402, 2.500000000000000000, 6.595190528383296780 ) ) ;
#113355=DIRECTION ( 'NONE',  ( 0.000000000000000000, 1.000000000000000000, 0.000000000000000000 ) ) ;
#113356=AXIS2_PLACEMENT_3D ( 'NONE', #4397, #76403, #36496 ) ;
#113357=CARTESIAN_POINT ( 'NONE',  ( -9.150000000000005684, 2.500000000000000000, 6.495190528383297135 ) ) ;
#113358=CARTESIAN_POINT ( 'NONE',  ( 1.249999999999952038, 2.500000000000000000, 5.702370205355745014 ) ) ;
#113359=DIRECTION ( 'NONE',  ( 0.000000000000000000, -0.000000000000000000, 1.000000000000000000 ) ) ;
#113360=DIRECTION ( 'NONE',  ( 0.000000000000000000, 0.000000000000000000, 1.000000000000000000 ) ) ;
#113361=DIRECTION ( 'NONE',  ( 0.000000000000000000, 0.000000000000000000, -1.000000000000000000 ) ) ;
#113362=CARTESIAN_POINT ( 'NONE',  ( 4.599999999999940137, 2.500000000000000000, -5.122947341949753763 ) ) ;
#113363=ADVANCED_FACE ( 'NONE', ( #92374 ), #29249, .T. ) ;
#113365=CARTESIAN_POINT ( 'NONE',  ( -5.600000000000023626, 2.500000000000000000, -3.983716857408426293 ) ) ;
#113366=CARTESIAN_POINT ( 'NONE',  ( -7.950000000000012612, 2.500000000000000000, -2.165063509461101710 ) ) ;
#113367=ORIENTED_EDGE ( 'NONE', *, *, #85172, .T. ) ;
#113368=VERTEX_POINT ( 'NONE', #110723 ) ;
#113369=EDGE_LOOP ( 'NONE', ( #87677, #66599, #56013, #50435 ) ) ;
#113370=CARTESIAN_POINT ( 'NONE',  ( 3.149999999999942624, 2.500000000000000000, 6.148780366869520897 ) ) ;
#113371=ORIENTED_EDGE ( 'NONE', *, *, #60858, .F. ) ;
#113372=DIRECTION ( 'NONE',  ( 0.000000000000000000, 0.000000000000000000, 1.000000000000000000 ) ) ;
#113373=ORIENTED_EDGE ( 'NONE', *, *, #17549, .F. ) ;
#113374=ORIENTED_EDGE ( 'NONE', *, *, #104637, .F. ) ;
#113375=ORIENTED_EDGE ( 'NONE', *, *, #59596, .F. ) ;
#113376=DIRECTION ( 'NONE',  ( 0.000000000000000000, 0.000000000000000000, 1.000000000000000000 ) ) ;
#113377=VECTOR ( 'NONE', #21866, 1000.000000000000000 ) ;
#113378=PLANE ( 'NONE',  #9168 ) ;
#113379=ADVANCED_FACE ( 'NONE', ( #89802 ), #96118, .T. ) ;
#113381=CARTESIAN_POINT ( 'NONE',  ( -4.400000000000025224, 2.500000000000000000, 0.3464101615137735735 ) ) ;
#113382=CARTESIAN_POINT ( 'NONE',  ( -7.700000000000012612, 2.500000000000000000, 4.776537180435972196 ) ) ;
#113383=ORIENTED_EDGE ( 'NONE', *, *, #123684, .T. ) ;
#113385=CIRCLE ( 'NONE', #6746, 0.06509327318403741736 ) ;
#113386=CARTESIAN_POINT ( 'NONE',  ( 9.349999999999916156, 12.50000000000000000, 6.776507416713035248 ) ) ;
#113387=ORIENTED_EDGE ( 'NONE', *, *, #172, .F. ) ;
#113388=CONICAL_SURFACE ( 'NONE', #125896, 0.1000000000000002554, 0.003490658503988666988 ) ;
#113389=EDGE_CURVE ( 'NONE', #4798, #85752, #1417, .T. ) ;
#113390=ORIENTED_EDGE ( 'NONE', *, *, #123893, .T. ) ;
#113391=VECTOR ( 'NONE', #112162, 1000.000000000000000 ) ;
#113392=ORIENTED_EDGE ( 'NONE', *, *, #100581, .T. ) ;
#113393=CARTESIAN_POINT ( 'NONE',  ( -15.59999999999998010, 12.50000000000000000, 0.3464101615137759604 ) ) ;
#113394=EDGE_CURVE ( 'NONE', #110762, #16380, #10444, .T. ) ;
#113395=VERTEX_POINT ( 'NONE', #12523 ) ;
#113396=EDGE_CURVE ( 'NONE', #50485, #96613, #54358, .T. ) ;
#113397=ORIENTED_EDGE ( 'NONE', *, *, #125677, .F. ) ;
#113398=EDGE_CURVE ( 'NONE', #28288, #62105, #119912, .T. ) ;
#113399=ORIENTED_EDGE ( 'NONE', *, *, #77240, .F. ) ;
#113400=ADVANCED_FACE ( 'NONE', ( #60373 ), #125461, .T. ) ;
#113401=DIRECTION ( 'NONE',  ( 0.000000000000000000, 1.000000000000000000, 0.000000000000000000 ) ) ;
#113402=CIRCLE ( 'NONE', #29877, 0.1000000000000002554 ) ;
#113404=DIRECTION ( 'NONE',  ( -4.274815082592931898E-19, -0.9999939076577903929, -0.003490651415223739937 ) ) ;
#113405=DIRECTION ( 'NONE',  ( 0.000000000000000000, 0.000000000000000000, -1.000000000000000000 ) ) ;
#113406=VECTOR ( 'NONE', #3920, 1000.000000000000000 ) ;
#113407=DIRECTION ( 'NONE',  ( 0.000000000000000000, 0.000000000000000000, 1.000000000000000000 ) ) ;
#113408=VECTOR ( 'NONE', #42593, 1000.000000000000000 ) ;
#113409=AXIS2_PLACEMENT_3D ( 'NONE', #95507, #94216, #104664 ) ;
#113410=ADVANCED_FACE ( 'NONE', ( #22376 ), #21055, .T. ) ;
#113411=DIRECTION ( 'NONE',  ( 0.000000000000000000, 1.000000000000000000, 0.000000000000000000 ) ) ;
#113412=EDGE_CURVE ( 'NONE', #128788, #78315, #10579, .T. ) ;
#113413=AXIS2_PLACEMENT_3D ( 'NONE', #45094, #117014, #105291 ) ;
#113414=FACE_OUTER_BOUND ( 'NONE', #71511, .T. ) ;
#113415=ORIENTED_EDGE ( 'NONE', *, *, #35112, .T. ) ;
#113416=LINE ( 'NONE', #23759, #123731 ) ;
#113417=ADVANCED_FACE ( 'NONE', ( #772 ), #117028, .T. ) ;
#113418=ORIENTED_EDGE ( 'NONE', *, *, #100636, .F. ) ;
#113419=AXIS2_PLACEMENT_3D ( 'NONE', #23514, #113844, #114473 ) ;
#113420=DIRECTION ( 'NONE',  ( 0.000000000000000000, -0.000000000000000000, 1.000000000000000000 ) ) ;
#113421=EDGE_LOOP ( 'NONE', ( #82066, #101240 ) ) ;
#113423=VERTEX_POINT ( 'NONE', #91096 ) ;
#113424=EDGE_CURVE ( 'NONE', #69423, #49637, #92018, .T. ) ;
#113425=DIRECTION ( 'NONE',  ( -0.000000000000000000, -1.000000000000000000, -0.000000000000000000 ) ) ;
#113426=DIRECTION ( 'NONE',  ( 0.000000000000000000, 1.000000000000000000, 0.000000000000000000 ) ) ;
#113427=DIRECTION ( 'NONE',  ( -0.000000000000000000, -1.000000000000000000, -0.000000000000000000 ) ) ;
#113428=EDGE_LOOP ( 'NONE', ( #29897, #48408 ) ) ;
#113429=ORIENTED_EDGE ( 'NONE', *, *, #71310, .F. ) ;
#113430=DIRECTION ( 'NONE',  ( 0.000000000000000000, 0.000000000000000000, -1.000000000000000000 ) ) ;
#113431=CARTESIAN_POINT ( 'NONE',  ( 1.049999999999953637, 2.500000000000000000, -1.718653347947326049 ) ) ;
#113432=CIRCLE ( 'NONE', #119679, 0.09999999999999982514 ) ;
#113433=PLANE ( 'NONE',  #2070 ) ;
#113434=DIRECTION ( 'NONE',  ( 0.000000000000000000, 0.000000000000000000, 1.000000000000000000 ) ) ;
#113435=CARTESIAN_POINT ( 'NONE',  ( 0.6499999999999561684, 2.500000000000000000, -1.718653347947325827 ) ) ;
#113436=EDGE_LOOP ( 'NONE', ( #102183, #129031 ) ) ;
#113437=CONICAL_SURFACE ( 'NONE', #21498, 0.1000000000000002554, 0.003490658503988666988 ) ;
#113438=VECTOR ( 'NONE', #32476, 1000.000000000000000 ) ;
#113439=EDGE_LOOP ( 'NONE', ( #9511, #109206, #55651, #98121 ) ) ;
#113440=FACE_OUTER_BOUND ( 'NONE', #80980, .T. ) ;
#113441=DIRECTION ( 'NONE',  ( 0.000000000000000000, 1.000000000000000000, 0.000000000000000000 ) ) ;
#113442=AXIS2_PLACEMENT_3D ( 'NONE', #121769, #92312, #70749 ) ;
#113443=AXIS2_PLACEMENT_3D ( 'NONE', #16017, #65115, #116156 ) ;
#113444=CONICAL_SURFACE ( 'NONE', #29832, 0.09999999999999982514, 0.003490658503988666988 ) ;
#113445=AXIS2_PLACEMENT_3D ( 'NONE', #99717, #55430, #40147 ) ;
#113447=DIRECTION ( 'NONE',  ( -0.000000000000000000, 1.000000000000000000, -0.000000000000000000 ) ) ;
#113448=DIRECTION ( 'NONE',  ( -0.000000000000000000, 1.000000000000000000, -0.000000000000000000 ) ) ;
#113449=DIRECTION ( 'NONE',  ( -0.000000000000000000, -1.000000000000000000, -0.000000000000000000 ) ) ;
#113450=CARTESIAN_POINT ( 'NONE',  ( 5.399999999999934630, 12.50000000000000000, -0.6928203230275542523 ) ) ;
#113451=ORIENTED_EDGE ( 'NONE', *, *, #2067, .T. ) ;
#113452=AXIS2_PLACEMENT_3D ( 'NONE', #52732, #53391, #122135 ) ;
#113453=DIRECTION ( 'NONE',  ( 0.000000000000000000, 1.000000000000000000, 0.000000000000000000 ) ) ;
#113454=ADVANCED_FACE ( 'NONE', ( #121193 ), #6217, .T. ) ;
#113455=CARTESIAN_POINT ( 'NONE',  ( -13.34999999999999076, 2.500000000000000000, 1.472243186433549456 ) ) ;
#113456=DIRECTION ( 'NONE',  ( 0.000000000000000000, 0.000000000000000000, 1.000000000000000000 ) ) ;
#113457=ADVANCED_FACE ( 'NONE', ( #61649 ), #22978, .T. ) ;
#113458=ORIENTED_EDGE ( 'NONE', *, *, #2884, .F. ) ;
#113459=CARTESIAN_POINT ( 'NONE',  ( 6.849999999999929479, 12.50000000000000000, 6.148780366869520009 ) ) ;
#113460=CIRCLE ( 'NONE', #75799, 0.06509327318403741736 ) ;
#113461=ORIENTED_EDGE ( 'NONE', *, *, #95925, .T. ) ;
#113462=CARTESIAN_POINT ( 'NONE',  ( -8.150000000000012790, 2.500000000000000000, 2.411473670974873862 ) ) ;
#113463=ORIENTED_EDGE ( 'NONE', *, *, #12466, .T. ) ;
#113464=DIRECTION ( 'NONE',  ( -4.274815082592931898E-19, -0.9999939076577903929, -0.003490651415223739937 ) ) ;
#113465=DIRECTION ( 'NONE',  ( 0.000000000000000000, 0.000000000000000000, 1.000000000000000000 ) ) ;
#113466=FACE_OUTER_BOUND ( 'NONE', #66729, .T. ) ;
#113467=AXIS2_PLACEMENT_3D ( 'NONE', #123273, #4121, #93183 ) ;
#113468=ORIENTED_EDGE ( 'NONE', *, *, #63612, .T. ) ;
#113469=AXIS2_PLACEMENT_3D ( 'NONE', #59916, #67093, #88705 ) ;
#113470=AXIS2_PLACEMENT_3D ( 'NONE', #116560, #34154, #26904 ) ;
#113471=CARTESIAN_POINT ( 'NONE',  ( 7.499999999999927169, 2.500000000000000000, -5.122947341949753763 ) ) ;
#113472=DIRECTION ( 'NONE',  ( 0.000000000000000000, -0.9999939076577903929, 0.003490651415223739937 ) ) ;
#113473=ORIENTED_EDGE ( 'NONE', *, *, #53289, .T. ) ;
#113474=CIRCLE ( 'NONE', #54986, 0.06509327318403745899 ) ;
#113475=AXIS2_PLACEMENT_3D ( 'NONE', #57005, #96937, #55094 ) ;
#113476=ORIENTED_EDGE ( 'NONE', *, *, #56547, .T. ) ;
#113477=VERTEX_POINT ( 'NONE', #105433 ) ;
#113478=CARTESIAN_POINT ( 'NONE',  ( 11.64999999999990621, 12.50000000000000000, -2.165063509461101710 ) ) ;
#113479=CARTESIAN_POINT ( 'NONE',  ( 7.899999999999921307, 12.50000000000000000, -2.385244779468109755E-15 ) ) ;
#113480=DIRECTION ( 'NONE',  ( 0.000000000000000000, 0.000000000000000000, -1.000000000000000000 ) ) ;
#113481=VERTEX_POINT ( 'NONE', #62923 ) ;
#113482=CARTESIAN_POINT ( 'NONE',  ( -8.350000000000012079, 2.500000000000000000, 2.757883832488649656 ) ) ;
#113483=DIRECTION ( 'NONE',  ( -0.000000000000000000, 1.000000000000000000, -0.000000000000000000 ) ) ;
#113485=LINE ( 'NONE', #63100, #34234 ) ;
#113486=EDGE_CURVE ( 'NONE', #31178, #97758, #106583, .T. ) ;
#113487=DIRECTION ( 'NONE',  ( -0.000000000000000000, 1.000000000000000000, -0.000000000000000000 ) ) ;
#113488=CONICAL_SURFACE ( 'NONE', #105174, 0.1000000000000002554, 0.003490658503988666988 ) ;
#113489=CONICAL_SURFACE ( 'NONE', #46596, 0.1000000000000002554, 0.003490658503988666988 ) ;
#113490=VECTOR ( 'NONE', #3115, 1000.000000000000000 ) ;
#113491=FACE_OUTER_BOUND ( 'NONE', #19656, .T. ) ;
#113492=CARTESIAN_POINT ( 'NONE',  ( 0.8499999999999527933, 12.50000000000000000, 7.122917578226811486 ) ) ;
#113493=DIRECTION ( 'NONE',  ( 0.000000000000000000, 1.000000000000000000, 0.000000000000000000 ) ) ;
#113494=DIRECTION ( 'NONE',  ( 0.000000000000000000, 1.000000000000000000, 0.000000000000000000 ) ) ;
#113495=VECTOR ( 'NONE', #124775, 1000.000000000000000 ) ;
#113496=DIRECTION ( 'NONE',  ( -0.000000000000000000, -1.000000000000000000, -0.000000000000000000 ) ) ;
#113497=VERTEX_POINT ( 'NONE', #104755 ) ;
#113498=CIRCLE ( 'NONE', #82112, 0.1000000000000002554 ) ;
#113499=ORIENTED_EDGE ( 'NONE', *, *, #15275, .T. ) ;
#113500=ORIENTED_EDGE ( 'NONE', *, *, #101081, .T. ) ;
#113501=VERTEX_POINT ( 'NONE', #55035 ) ;
#113502=DIRECTION ( 'NONE',  ( -4.274815082592931898E-19, -0.9999939076577903929, -0.003490651415223739937 ) ) ;
#113503=CARTESIAN_POINT ( 'NONE',  ( -6.850000000000013856, 12.50000000000000000, 1.818653347947321475 ) ) ;
#113504=EDGE_CURVE ( 'NONE', #126044, #23819, #73147, .T. ) ;
#113505=DIRECTION ( 'NONE',  ( 0.000000000000000000, 0.000000000000000000, -1.000000000000000000 ) ) ;
#113506=VERTEX_POINT ( 'NONE', #5279 ) ;
#113507=FACE_BOUND ( 'NONE', #5455, .T. ) ;
#113508=ADVANCED_FACE ( 'NONE', ( #85772 ), #115886, .T. ) ;
#113509=DIRECTION ( 'NONE',  ( 0.000000000000000000, 0.000000000000000000, 1.000000000000000000 ) ) ;
#113510=DIRECTION ( 'NONE',  ( 0.000000000000000000, -0.9999939076577903929, 0.003490651415223739937 ) ) ;
#113511=DIRECTION ( 'NONE',  ( 0.000000000000000000, 0.000000000000000000, 1.000000000000000000 ) ) ;
#113512=CARTESIAN_POINT ( 'NONE',  ( -8.300000000000011369, 2.500000000000000000, 0.09999999999999772959 ) ) ;
#113513=DIRECTION ( 'NONE',  ( 0.000000000000000000, 0.000000000000000000, 1.000000000000000000 ) ) ;
#113514=CARTESIAN_POINT ( 'NONE',  ( 2.949999999999946887, 2.500000000000000000, -2.065063509461102065 ) ) ;
#113515=FACE_OUTER_BOUND ( 'NONE', #5674, .T. ) ;
#113516=CARTESIAN_POINT ( 'NONE',  ( -9.550000000000007816, 12.50000000000000000, -6.495190528383297135 ) ) ;
#113517=AXIS2_PLACEMENT_3D ( 'NONE', #114513, #72037, #124354 ) ;
#113518=VECTOR ( 'NONE', #31999, 1000.000000000000000 ) ;
#113519=ADVANCED_FACE ( 'NONE', ( #115210 ), #35592, .T. ) ;
#113520=LINE ( 'NONE', #51408, #70571 ) ;
#113521=DIRECTION ( 'NONE',  ( -0.000000000000000000, -1.000000000000000000, -0.000000000000000000 ) ) ;
#113522=ORIENTED_EDGE ( 'NONE', *, *, #102232, .T. ) ;
#113523=CONICAL_SURFACE ( 'NONE', #2695, 0.1000000000000002554, 0.003490658503988666988 ) ;
#113524=ORIENTED_EDGE ( 'NONE', *, *, #71949, .T. ) ;
#113525=ORIENTED_EDGE ( 'NONE', *, *, #46925, .T. ) ;
#113526=ORIENTED_EDGE ( 'NONE', *, *, #90945, .T. ) ;
#113527=AXIS2_PLACEMENT_3D ( 'NONE', #77277, #108018, #68743 ) ;
#113528=ORIENTED_EDGE ( 'NONE', *, *, #95935, .F. ) ;
#113530=EDGE_LOOP ( 'NONE', ( #40536, #26317 ) ) ;
#113531=VECTOR ( 'NONE', #7484, 1000.000000000000000 ) ;
#113532=CARTESIAN_POINT ( 'NONE',  ( -5.650000000000023448, 12.50000000000000000, -1.883746621131363597 ) ) ;
#113533=VERTEX_POINT ( 'NONE', #15078 ) ;
#113534=VERTEX_POINT ( 'NONE', #103500 ) ;
#113535=VECTOR ( 'NONE', #59706, 1000.000000000000000 ) ;
#113536=CIRCLE ( 'NONE', #19434, 0.06509327318403745899 ) ;
#113537=CARTESIAN_POINT ( 'NONE',  ( 16.04744069018120811, -1.500000000000000222, 6.586254744913174974 ) ) ;
#113539=DIRECTION ( 'NONE',  ( 0.000000000000000000, 0.000000000000000000, 1.000000000000000000 ) ) ;
#113540=CIRCLE ( 'NONE', #6899, 0.1000000000000002554 ) ;
#113541=CONICAL_SURFACE ( 'NONE', #6902, 0.1000000000000002554, 0.003490658503988666988 ) ;
#113542=EDGE_LOOP ( 'NONE', ( #31882, #48033, #87594, #71672 ) ) ;
#113543=FACE_OUTER_BOUND ( 'NONE', #18661, .T. ) ;
#113544=VECTOR ( 'NONE', #7324, 1000.000000000000000 ) ;
#113545=ORIENTED_EDGE ( 'NONE', *, *, #82555, .F. ) ;
#113546=EDGE_CURVE ( 'NONE', #72199, #83267, #52309, .T. ) ;
#113547=EDGE_LOOP ( 'NONE', ( #113660, #121652 ) ) ;
#113548=LINE ( 'NONE', #63813, #99147 ) ;
#113549=EDGE_LOOP ( 'NONE', ( #40743, #116226 ) ) ;
#113550=FACE_OUTER_BOUND ( 'NONE', #66142, .T. ) ;
#113551=ADVANCED_FACE ( 'NONE', ( #24936 ), #36050, .T. ) ;
#113554=ADVANCED_FACE ( 'NONE', ( #83841 ), #66872, .T. ) ;
#113555=CONICAL_SURFACE ( 'NONE', #82166, 0.1000000000000002554, 0.003490658503988666988 ) ;
#113556=DIRECTION ( 'NONE',  ( 0.000000000000000000, 0.000000000000000000, 1.000000000000000000 ) ) ;
#113557=FACE_OUTER_BOUND ( 'NONE', #33006, .T. ) ;
#113558=DIRECTION ( 'NONE',  ( -0.000000000000000000, -1.000000000000000000, -0.000000000000000000 ) ) ;
#113559=CARTESIAN_POINT ( 'NONE',  ( -3.550000000000028688, 2.500000000000000000, 6.841600689897072485 ) ) ;
#113560=EDGE_CURVE ( 'NONE', #124307, #119121, #77350, .T. ) ;
#113561=ADVANCED_FACE ( 'NONE', ( #102832 ), #13156, .T. ) ;
#113562=CARTESIAN_POINT ( 'NONE',  ( -7.700000000000012612, 12.50000000000000000, 4.741630453620009789 ) ) ;
#113563=EDGE_CURVE ( 'NONE', #93080, #69989, #93038, .T. ) ;
#113564=EDGE_CURVE ( 'NONE', #29080, #92178, #27167, .T. ) ;
#113565=EDGE_CURVE ( 'NONE', #116268, #85461, #100340, .T. ) ;
#113566=AXIS2_PLACEMENT_3D ( 'NONE', #37166, #8321, #88154 ) ;
#113567=ORIENTED_EDGE ( 'NONE', *, *, #81293, .T. ) ;
#113568=CARTESIAN_POINT ( 'NONE',  ( 7.499999999999961808, 12.50000000000000000, -4.330127018922201643 ) ) ;
#113569=VECTOR ( 'NONE', #105619, 1000.000000000000000 ) ;
#113570=CONICAL_SURFACE ( 'NONE', #25730, 0.1000000000000002554, 0.003490658503988666988 ) ;
#113571=ORIENTED_EDGE ( 'NONE', *, *, #3505, .T. ) ;
#113572=FACE_OUTER_BOUND ( 'NONE', #42371, .T. ) ;
#113573=ADVANCED_FACE ( 'NONE', ( #23644 ), #71090, .T. ) ;
#113574=EDGE_LOOP ( 'NONE', ( #83586, #129056 ) ) ;
#113575=DIRECTION ( 'NONE',  ( 0.000000000000000000, 0.000000000000000000, 1.000000000000000000 ) ) ;
#113576=FACE_OUTER_BOUND ( 'NONE', #23049, .T. ) ;
#113577=CARTESIAN_POINT ( 'NONE',  ( 4.999999999999971578, 2.500000000000000000, -0.1000000000000022815 ) ) ;
#113578=CARTESIAN_POINT ( 'NONE',  ( 11.24999999999990763, 2.500000000000000000, -7.088010851410853519 ) ) ;
#113579=CONICAL_SURFACE ( 'NONE', #25844, 0.1000000000000002554, 0.003490658503988666988 ) ;
#113581=AXIS2_PLACEMENT_3D ( 'NONE', #1198, #11661, #43730 ) ;
#113582=EDGE_CURVE ( 'NONE', #27024, #47911, #4165, .T. ) ;
#113583=CIRCLE ( 'NONE', #109373, 0.1000000000000000056 ) ;
#113584=DIRECTION ( 'NONE',  ( 0.000000000000000000, 0.000000000000000000, 1.000000000000000000 ) ) ;
#113585=AXIS2_PLACEMENT_3D ( 'NONE', #55653, #95586, #5887 ) ;
#113586=DIRECTION ( 'NONE',  ( 0.000000000000000000, 0.000000000000000000, -1.000000000000000000 ) ) ;
#113587=ORIENTED_EDGE ( 'NONE', *, *, #48913, .T. ) ;
#113588=ORIENTED_EDGE ( 'NONE', *, *, #93150, .T. ) ;
#113589=VERTEX_POINT ( 'NONE', #74036 ) ;
#113590=DIRECTION ( 'NONE',  ( 0.000000000000000000, 0.000000000000000000, -1.000000000000000000 ) ) ;
#113591=DIRECTION ( 'NONE',  ( 0.000000000000000000, 1.000000000000000000, 0.000000000000000000 ) ) ;
#113593=DIRECTION ( 'NONE',  ( -0.000000000000000000, -1.000000000000000000, -0.000000000000000000 ) ) ;
#113594=CARTESIAN_POINT ( 'NONE',  ( 17.49149623775394602, 2.499999999999960920, -4.292098716152958460 ) ) ;
#113595=AXIS2_PLACEMENT_3D ( 'NONE', #2885, #33001, #42837 ) ;
#113596=CIRCLE ( 'NONE', #94810, 0.06509327318403745899 ) ;
#113597=FACE_OUTER_BOUND ( 'NONE', #9804, .T. ) ;
#113599=DIRECTION ( 'NONE',  ( 0.000000000000000000, 1.000000000000000000, 0.000000000000000000 ) ) ;
#113600=EDGE_LOOP ( 'NONE', ( #11099, #29636 ) ) ;
#113601=DIRECTION ( 'NONE',  ( 0.000000000000000000, 1.000000000000000000, 0.000000000000000000 ) ) ;
#113602=FACE_OUTER_BOUND ( 'NONE', #101022, .T. ) ;
#113604=DIRECTION ( 'NONE',  ( 0.000000000000000000, 0.000000000000000000, 1.000000000000000000 ) ) ;
#113605=EDGE_LOOP ( 'NONE', ( #38721, #128381, #25308, #119551 ) ) ;
#113606=EDGE_CURVE ( 'NONE', #26142, #30816, #87796, .T. ) ;
#113607=CARTESIAN_POINT ( 'NONE',  ( 4.549999999999939426, 2.500000000000000000, -2.165063509461101710 ) ) ;
#113608=DIRECTION ( 'NONE',  ( 0.000000000000000000, -0.9999939076577903929, 0.003490651415223739937 ) ) ;
#113609=ORIENTED_EDGE ( 'NONE', *, *, #103718, .T. ) ;
#113610=AXIS2_PLACEMENT_3D ( 'NONE', #28083, #94885, #96165 ) ;
#113611=AXIS2_PLACEMENT_3D ( 'NONE', #69095, #6929, #88068 ) ;
#113612=ORIENTED_EDGE ( 'NONE', *, *, #102904, .T. ) ;
#113613=CARTESIAN_POINT ( 'NONE',  ( 6.649999999999931966, 12.50000000000000000, -7.188010851410854052 ) ) ;
#113614=ADVANCED_FACE ( 'NONE', ( #26230 ), #36704, .T. ) ;
#113615=CONICAL_SURFACE ( 'NONE', #73808, 0.1000000000000002554, 0.003490658503988666988 ) ;
#113616=VECTOR ( 'NONE', #78662, 1000.000000000000000 ) ;
#113617=ORIENTED_EDGE ( 'NONE', *, *, #110853, .F. ) ;
#113618=CONICAL_SURFACE ( 'NONE', #59264, 0.09999999999999982514, 0.003490658503988666988 ) ;
#113619=EDGE_LOOP ( 'NONE', ( #63438, #67450 ) ) ;
#113620=LINE ( 'NONE', #95276, #27838 ) ;
#113621=AXIS2_PLACEMENT_3D ( 'NONE', #95359, #103887, #66524 ) ;
#113622=CONICAL_SURFACE ( 'NONE', #6990, 0.09999999999999982514, 0.003490658503988666988 ) ;
#113623=ORIENTED_EDGE ( 'NONE', *, *, #34, .F. ) ;
#113624=CARTESIAN_POINT ( 'NONE',  ( 16.58100817950494843, 2.557139044001659478, -6.067820687733441076 ) ) ;
#113625=DIRECTION ( 'NONE',  ( 0.000000000000000000, 0.000000000000000000, 1.000000000000000000 ) ) ;
#113626=LINE ( 'NONE', #52765, #77125 ) ;
#113627=CIRCLE ( 'NONE', #115672, 0.06509327318403745899 ) ;
#113628=ORIENTED_EDGE ( 'NONE', *, *, #127740, .T. ) ;
#113629=AXIS2_PLACEMENT_3D ( 'NONE', #61730, #102913, #13883 ) ;
#113630=AXIS2_PLACEMENT_3D ( 'NONE', #15920, #44765, #84674 ) ;
#113631=LINE ( 'NONE', #23965, #81711 ) ;
#113633=VERTEX_POINT ( 'NONE', #87708 ) ;
#113634=AXIS2_PLACEMENT_3D ( 'NONE', #4551, #53056, #23580 ) ;
#113635=DIRECTION ( 'NONE',  ( 0.000000000000000000, -0.000000000000000000, 1.000000000000000000 ) ) ;
#113636=DIRECTION ( 'NONE',  ( 0.000000000000000000, 1.000000000000000000, 0.000000000000000000 ) ) ;
#113637=VERTEX_POINT ( 'NONE', #106701 ) ;
#113638=EDGE_LOOP ( 'NONE', ( #8358, #118631 ) ) ;
#113639=ORIENTED_EDGE ( 'NONE', *, *, #31681, .F. ) ;
#113640=ORIENTED_EDGE ( 'NONE', *, *, #34157, .T. ) ;
#113641=CARTESIAN_POINT ( 'NONE',  ( -3.550000000000028688, 12.50000000000000000, 6.841600689897072485 ) ) ;
#113642=DIRECTION ( 'NONE',  ( -0.000000000000000000, -1.000000000000000000, -0.000000000000000000 ) ) ;
#113645=FACE_BOUND ( 'NONE', #117169, .T. ) ;
#113646=ORIENTED_EDGE ( 'NONE', *, *, #68950, .F. ) ;
#113648=FACE_OUTER_BOUND ( 'NONE', #75425, .T. ) ;
#113649=CARTESIAN_POINT ( 'NONE',  ( 11.04999999999991012, 12.50000000000000000, 6.841600689897072485 ) ) ;
#113650=CIRCLE ( 'NONE', #2837, 0.06509327318403745899 ) ;
#113652=CARTESIAN_POINT ( 'NONE',  ( 6.649999999999931077, 2.500000000000000000, -6.495190528383302464 ) ) ;
#113653=CARTESIAN_POINT ( 'NONE',  ( 3.949999999999938005, 12.50000000000000000, 6.906693963081109722 ) ) ;
#113654=LINE ( 'NONE', #61988, #103473 ) ;
#113655=AXIS2_PLACEMENT_3D ( 'NONE', #122801, #45539, #22683 ) ;
#113656=CIRCLE ( 'NONE', #65528, 0.06509327318403745899 ) ;
#113657=EDGE_CURVE ( 'NONE', #82898, #76941, #64818, .T. ) ;
#113658=AXIS2_PLACEMENT_3D ( 'NONE', #8178, #68391, #126680 ) ;
#113660=ORIENTED_EDGE ( 'NONE', *, *, #60713, .F. ) ;
#113661=ORIENTED_EDGE ( 'NONE', *, *, #11123, .F. ) ;
#113662=ORIENTED_EDGE ( 'NONE', *, *, #123008, .T. ) ;
#113663=VERTEX_POINT ( 'NONE', #86420 ) ;
#113664=ORIENTED_EDGE ( 'NONE', *, *, #115408, .F. ) ;
#113665=DIRECTION ( 'NONE',  ( 0.000000000000000000, 0.000000000000000000, 1.000000000000000000 ) ) ;
#113666=EDGE_CURVE ( 'NONE', #11828, #76998, #98267, .T. ) ;
#113667=DIRECTION ( 'NONE',  ( -0.000000000000000000, -1.000000000000000000, -0.000000000000000000 ) ) ;
#113668=EDGE_LOOP ( 'NONE', ( #26683, #15957, #26993, #124007 ) ) ;
#113669=FACE_BOUND ( 'NONE', #28483, .T. ) ;
#113670=AXIS2_PLACEMENT_3D ( 'NONE', #39781, #453, #8994 ) ;
#113672=AXIS2_PLACEMENT_3D ( 'NONE', #61267, #31806, #41645 ) ;
#113673=FACE_OUTER_BOUND ( 'NONE', #4701, .T. ) ;
#113674=CIRCLE ( 'NONE', #57234, 0.1000000000000002554 ) ;
#113676=EDGE_CURVE ( 'NONE', #19759, #113210, #83988, .T. ) ;
#113677=ORIENTED_EDGE ( 'NONE', *, *, #13068, .T. ) ;
#113678=DIRECTION ( 'NONE',  ( -0.000000000000000000, 1.000000000000000000, -0.000000000000000000 ) ) ;
#113679=LINE ( 'NONE', #52179, #115800 ) ;
#113680=EDGE_CURVE ( 'NONE', #49878, #59844, #26868, .T. ) ;
#113681=DIRECTION ( 'NONE',  ( 0.000000000000000000, 0.000000000000000000, 1.000000000000000000 ) ) ;
#113682=CIRCLE ( 'NONE', #51001, 0.06509327318403745899 ) ;
#113683=ORIENTED_EDGE ( 'NONE', *, *, #32597, .T. ) ;
#113684=FACE_OUTER_BOUND ( 'NONE', #23022, .T. ) ;
#113685=ORIENTED_EDGE ( 'NONE', *, *, #96861, .T. ) ;
#113686=AXIS2_PLACEMENT_3D ( 'NONE', #26398, #105600, #66302 ) ;
#113687=AXIS2_PLACEMENT_3D ( 'NONE', #89910, #108891, #78173 ) ;
#113688=ORIENTED_EDGE ( 'NONE', *, *, #3767, .F. ) ;
#113689=VERTEX_POINT ( 'NONE', #116526 ) ;
#113690=CARTESIAN_POINT ( 'NONE',  ( -11.25000000000000000, 12.50000000000000000, 2.857883832488649301 ) ) ;
#113692=DIRECTION ( 'NONE',  ( 0.000000000000000000, 0.000000000000000000, -1.000000000000000000 ) ) ;
#113693=AXIS2_PLACEMENT_3D ( 'NONE', #10001, #17877, #108188 ) ;
#113694=ORIENTED_EDGE ( 'NONE', *, *, #63324, .F. ) ;
#113695=DIRECTION ( 'NONE',  ( -0.000000000000000000, 1.000000000000000000, -0.000000000000000000 ) ) ;
#113696=VECTOR ( 'NONE', #115389, 1000.000000000000000 ) ;
#113697=DIRECTION ( 'NONE',  ( -0.000000000000000000, -1.000000000000000000, -0.000000000000000000 ) ) ;
#113698=CARTESIAN_POINT ( 'NONE',  ( 2.499999999999947153, 12.50000000000000000, 0.6928203230275494784 ) ) ;
#113700=ORIENTED_EDGE ( 'NONE', *, *, #38869, .T. ) ;
#113701=FACE_OUTER_BOUND ( 'NONE', #60609, .T. ) ;
#113702=ORIENTED_EDGE ( 'NONE', *, *, #5535, .F. ) ;
#113704=VERTEX_POINT ( 'NONE', #67401 ) ;
#113705=VERTEX_POINT ( 'NONE', #46495 ) ;
#113706=CARTESIAN_POINT ( 'NONE',  ( -5.850000000000019185, 2.500000000000000000, 6.495190528383297135 ) ) ;
#113707=CARTESIAN_POINT ( 'NONE',  ( 9.999999999999948486, 2.500000000000000000, 4.330127018922196314 ) ) ;
#113708=CIRCLE ( 'NONE', #111550, 0.06509327318403745899 ) ;
#113709=FACE_OUTER_BOUND ( 'NONE', #39002, .T. ) ;
#113710=VECTOR ( 'NONE', #17560, 1000.000000000000000 ) ;
#113711=CARTESIAN_POINT ( 'NONE',  ( 5.399999999999934630, 2.500000000000000000, -0.7928203230275543412 ) ) ;
#113713=ORIENTED_EDGE ( 'NONE', *, *, #110310, .F. ) ;
#113714=ORIENTED_EDGE ( 'NONE', *, *, #76389, .F. ) ;
#113716=AXIS2_PLACEMENT_3D ( 'NONE', #36369, #116827, #26529 ) ;
#113717=CONICAL_SURFACE ( 'NONE', #80273, 0.1000000000000002554, 0.003490658503988666988 ) ;
#113718=CONICAL_SURFACE ( 'NONE', #109513, 0.1000000000000000472, 0.003490658503988666988 ) ;
#113719=CARTESIAN_POINT ( 'NONE',  ( 0.5999999999999551248, 2.500000000000000000, -4.776537180435978414 ) ) ;
#113720=CONICAL_SURFACE ( 'NONE', #57282, 0.1000000000000002554, 0.003490658503988666988 ) ;
#113721=CARTESIAN_POINT ( 'NONE',  ( -5.600000000000020073, 2.500000000000000000, 3.883716857408421319 ) ) ;
#113722=ADVANCED_FACE ( 'NONE', ( #38647 ), #66777, .T. ) ;
#113723=ORIENTED_EDGE ( 'NONE', *, *, #70162, .T. ) ;
#113724=ORIENTED_EDGE ( 'NONE', *, *, #33492, .F. ) ;
#113725=ADVANCED_FACE ( 'NONE', ( #49104 ), #56314, .T. ) ;
#113726=DIRECTION ( 'NONE',  ( 0.000000000000000000, 1.000000000000000000, 0.000000000000000000 ) ) ;
#113727=EDGE_CURVE ( 'NONE', #46092, #116053, #17678, .T. ) ;
#113728=EDGE_CURVE ( 'NONE', #44827, #86121, #65116, .T. ) ;
#113729=ORIENTED_EDGE ( 'NONE', *, *, #93828, .T. ) ;
#113730=DIRECTION ( 'NONE',  ( -0.000000000000000000, 1.000000000000000000, -0.000000000000000000 ) ) ;
#113731=AXIS2_PLACEMENT_3D ( 'NONE', #109921, #71266, #52285 ) ;
#113732=AXIS2_PLACEMENT_3D ( 'NONE', #63513, #104699, #103434 ) ;
#113733=AXIS2_PLACEMENT_3D ( 'NONE', #126386, #54410, #116553 ) ;
#113734=CARTESIAN_POINT ( 'NONE',  ( -11.44999999999999929, 2.500000000000000000, -1.818653347947322141 ) ) ;
#113736=DIRECTION ( 'NONE',  ( -0.000000000000000000, 1.000000000000000000, -0.000000000000000000 ) ) ;
#113737=EDGE_CURVE ( 'NONE', #13514, #46605, #87064, .T. ) ;
#113738=CARTESIAN_POINT ( 'NONE',  ( -8.350000000000010303, 2.500000000000000000, 6.395190528383296602 ) ) ;
#113739=DIRECTION ( 'NONE',  ( 0.000000000000000000, -0.9999939076577903929, 0.003490651415223739937 ) ) ;
#113740=AXIS2_PLACEMENT_3D ( 'NONE', #27435, #97480, #68017 ) ;
#113741=FACE_OUTER_BOUND ( 'NONE', #99625, .T. ) ;
#113743=EDGE_CURVE ( 'NONE', #32290, #31868, #98556, .T. ) ;
#113744=CARTESIAN_POINT ( 'NONE',  ( 10.84999999999990905, 2.500000000000000000, -6.395190528383301931 ) ) ;
#113745=EDGE_CURVE ( 'NONE', #22907, #114764, #75586, .T. ) ;
#113746=DIRECTION ( 'NONE',  ( -0.000000000000000000, 1.000000000000000000, -0.000000000000000000 ) ) ;
#113747=CONICAL_SURFACE ( 'NONE', #100912, 0.1000000000000000472, 0.003490658503988666988 ) ;
#113748=ORIENTED_EDGE ( 'NONE', *, *, #118887, .T. ) ;
#113749=VERTEX_POINT ( 'NONE', #47806 ) ;
#113751=CARTESIAN_POINT ( 'NONE',  ( 7.699999999999925571, 12.50000000000000000, -4.741630453620016006 ) ) ;
#113752=CARTESIAN_POINT ( 'NONE',  ( -7.900000000000014566, 2.500000000000000000, -0.6928203230275541413 ) ) ;
#113753=AXIS2_PLACEMENT_3D ( 'NONE', #117154, #105434, #5280 ) ;
#113754=CARTESIAN_POINT ( 'NONE',  ( -12.29999999999999538, 12.50000000000000000, -4.611443907251937979 ) ) ;
#113755=DIRECTION ( 'NONE',  ( 0.000000000000000000, 1.000000000000000000, 0.000000000000000000 ) ) ;
#113756=DIRECTION ( 'NONE',  ( 0.000000000000000000, -0.9999939076577903929, 0.003490651415223739937 ) ) ;
#113757=CARTESIAN_POINT ( 'NONE',  ( -13.74999999999998757, 2.500000000000000000, 1.572243186433549544 ) ) ;
#113758=CARTESIAN_POINT ( 'NONE',  ( 1.849999999999950129, 2.500000000000000000, -6.841600689897078702 ) ) ;
#113759=CARTESIAN_POINT ( 'NONE',  ( -12.09999999999999609, 12.50000000000000000, -4.330127018922198978 ) ) ;
#113760=FACE_OUTER_BOUND ( 'NONE', #49510, .T. ) ;
#113761=CARTESIAN_POINT ( 'NONE',  ( -1.050000000000038236, 2.500000000000000000, -6.248780366869526759 ) ) ;
#113762=AXIS2_PLACEMENT_3D ( 'NONE', #53774, #125094, #93703 ) ;
#113764=CONICAL_SURFACE ( 'NONE', #32207, 0.09999999999999982514, 0.003490658503988666988 ) ;
#113765=EDGE_LOOP ( 'NONE', ( #112267, #21474 ) ) ;
#113766=EDGE_LOOP ( 'NONE', ( #86824, #129380 ) ) ;
#113767=ORIENTED_EDGE ( 'NONE', *, *, #16899, .F. ) ;
#113768=CARTESIAN_POINT ( 'NONE',  ( 13.29999999999990301, 12.50000000000000000, -4.265033745738164406 ) ) ;
#113769=LINE ( 'NONE', #117427, #58496 ) ;
#113770=ORIENTED_EDGE ( 'NONE', *, *, #25401, .T. ) ;
#113771=CARTESIAN_POINT ( 'NONE',  ( -12.94999999999999218, 12.50000000000000000, 2.230156782645138946 ) ) ;
#113772=VECTOR ( 'NONE', #19261, 1000.000000000000000 ) ;
#113773=CARTESIAN_POINT ( 'NONE',  ( 8.349999999999923261, 12.50000000000000000, -7.122917578226816815 ) ) ;
#113774=LINE ( 'NONE', #22826, #13987 ) ;
#113775=ORIENTED_EDGE ( 'NONE', *, *, #59366, .T. ) ;
#113776=CARTESIAN_POINT ( 'NONE',  ( -12.09999999999999609, 2.500000000000000000, -0.6928203230275501445 ) ) ;
#113777=FACE_OUTER_BOUND ( 'NONE', #2245, .T. ) ;
#113778=VERTEX_POINT ( 'NONE', #68073 ) ;
#113779=EDGE_CURVE ( 'NONE', #21428, #32421, #33826, .T. ) ;
#113780=CIRCLE ( 'NONE', #26040, 0.06509327318403745899 ) ;
#113781=CIRCLE ( 'NONE', #82399, 0.06509327318403745899 ) ;
#113782=ORIENTED_EDGE ( 'NONE', *, *, #124215, .F. ) ;
#113783=ORIENTED_EDGE ( 'NONE', *, *, #114850, .T. ) ;
#113784=ORIENTED_EDGE ( 'NONE', *, *, #89307, .T. ) ;
#113785=CARTESIAN_POINT ( 'NONE',  ( -4.999999999999986677, 2.500000000000000000, 4.430127018922196847 ) ) ;
#113786=AXIS2_PLACEMENT_3D ( 'NONE', #104177, #35449, #14484 ) ;
#113787=CARTESIAN_POINT ( 'NONE',  ( -0.4000000000000404898, 2.500000000000000000, 5.122947341949749323 ) ) ;
#113788=FACE_OUTER_BOUND ( 'NONE', #122944, .T. ) ;
#113789=VECTOR ( 'NONE', #93366, 1000.000000000000000 ) ;
#113790=DIRECTION ( 'NONE',  ( -0.000000000000000000, 1.000000000000000000, -0.000000000000000000 ) ) ;
#113791=ORIENTED_EDGE ( 'NONE', *, *, #97949, .T. ) ;
#113792=DIRECTION ( 'NONE',  ( 0.000000000000000000, 1.000000000000000000, 0.000000000000000000 ) ) ;
#113793=ORIENTED_EDGE ( 'NONE', *, *, #11878, .T. ) ;
#113794=DIRECTION ( 'NONE',  ( 0.000000000000000000, -0.000000000000000000, 1.000000000000000000 ) ) ;
#113795=CARTESIAN_POINT ( 'NONE',  ( 10.61495711640258932, -2.500000000000000888, -8.020491764208069085 ) ) ;
#113796=LINE ( 'NONE', #64045, #123700 ) ;
#113797=PLANE ( 'NONE',  #4501 ) ;
#113798=ORIENTED_EDGE ( 'NONE', *, *, #67748, .T. ) ;
#113799=CIRCLE ( 'NONE', #114083, 0.06509327318403741736 ) ;
#113800=ORIENTED_EDGE ( 'NONE', *, *, #13874, .F. ) ;
#113801=VECTOR ( 'NONE', #5704, 1000.000000000000000 ) ;
#113802=ORIENTED_EDGE ( 'NONE', *, *, #85171, .F. ) ;
#113803=CARTESIAN_POINT ( 'NONE',  ( -9.150000000000009237, 12.50000000000000000, 2.165063509461097713 ) ) ;
#113804=CARTESIAN_POINT ( 'NONE',  ( -12.94999999999999218, 12.50000000000000000, -2.165063509461099489 ) ) ;
#113805=CIRCLE ( 'NONE', #124268, 0.1000000000000000472 ) ;
#113806=CONICAL_SURFACE ( 'NONE', #57365, 0.1000000000000002554, 0.003490658503988666988 ) ;
#113807=CARTESIAN_POINT ( 'NONE',  ( -1.850000000000033840, 12.50000000000000000, 6.083687093685483660 ) ) ;
#113808=FACE_BOUND ( 'NONE', #123694, .T. ) ;
#113809=DIRECTION ( 'NONE',  ( 0.000000000000000000, 0.000000000000000000, -1.000000000000000000 ) ) ;
#113810=DIRECTION ( 'NONE',  ( 0.000000000000000000, 1.000000000000000000, 0.000000000000000000 ) ) ;
#113811=CARTESIAN_POINT ( 'NONE',  ( 0.000000000000000000, 2.500000000000000000, 9.000000000000001776 ) ) ;
#113812=AXIS2_PLACEMENT_3D ( 'NONE', #12287, #52234, #62703 ) ;
#113813=CIRCLE ( 'NONE', #936, 0.06509327318403745899 ) ;
#113815=CARTESIAN_POINT ( 'NONE',  ( -1.050000000000037348, 2.500000000000000000, -6.741600689897078169 ) ) ;
#113816=ORIENTED_EDGE ( 'NONE', *, *, #86413, .T. ) ;
#113817=CIRCLE ( 'NONE', #15506, 0.1000000000000002554 ) ;
#113818=CONICAL_SURFACE ( 'NONE', #101300, 0.09999999999999982514, 0.003490658503988666988 ) ;
#113819=EDGE_CURVE ( 'NONE', #93646, #81193, #68717, .T. ) ;
#113820=FACE_OUTER_BOUND ( 'NONE', #33009, .T. ) ;
#113821=EDGE_LOOP ( 'NONE', ( #21129, #113321 ) ) ;
#113822=ORIENTED_EDGE ( 'NONE', *, *, #73057, .F. ) ;
#113823=ORIENTED_EDGE ( 'NONE', *, *, #75693, .T. ) ;
#113824=EDGE_LOOP ( 'NONE', ( #36542, #39023, #52823, #93255 ) ) ;
#113825=AXIS2_PLACEMENT_3D ( 'NONE', #46956, #66563, #18113 ) ;
#113826=EDGE_CURVE ( 'NONE', #24484, #112609, #42152, .T. ) ;
#113827=CARTESIAN_POINT ( 'NONE',  ( 13.09999999999990195, 2.500000000000000000, 4.083716857408420609 ) ) ;
#113828=FACE_BOUND ( 'NONE', #20583, .T. ) ;
#113829=ADVANCED_FACE ( 'NONE', ( #19633 ), #11735, .T. ) ;
#113830=DIRECTION ( 'NONE',  ( -0.000000000000000000, 1.000000000000000000, -0.000000000000000000 ) ) ;
#113831=EDGE_CURVE ( 'NONE', #125498, #7881, #25402, .T. ) ;
#113832=ADVANCED_FACE ( 'NONE', ( #109290 ), #49752, .T. ) ;
#113833=ORIENTED_EDGE ( 'NONE', *, *, #82549, .F. ) ;
#113834=CARTESIAN_POINT ( 'NONE',  ( -8.100000000000013856, 12.50000000000000000, 0.4115034346978110880 ) ) ;
#113835=EDGE_CURVE ( 'NONE', #70628, #41760, #12875, .T. ) ;
#113836=EDGE_CURVE ( 'NONE', #81889, #51160, #100717, .T. ) ;
#113837=DIRECTION ( 'NONE',  ( 0.000000000000000000, 1.000000000000000000, 0.000000000000000000 ) ) ;
#113838=EDGE_CURVE ( 'NONE', #87808, #69735, #39925, .T. ) ;
#113839=AXIS2_PLACEMENT_3D ( 'NONE', #67613, #27065, #107559 ) ;
#113840=ORIENTED_EDGE ( 'NONE', *, *, #32447, .T. ) ;
#113841=DIRECTION ( 'NONE',  ( 0.000000000000000000, 0.000000000000000000, -1.000000000000000000 ) ) ;
#113842=DIRECTION ( 'NONE',  ( -0.000000000000000000, -1.000000000000000000, -0.000000000000000000 ) ) ;
#113843=ORIENTED_EDGE ( 'NONE', *, *, #120655, .F. ) ;
#113844=DIRECTION ( 'NONE',  ( 0.000000000000000000, 1.000000000000000000, 0.000000000000000000 ) ) ;
#113845=CARTESIAN_POINT ( 'NONE',  ( -5.850000000000018296, 2.500000000000000000, 5.902370205355745192 ) ) ;
#113846=EDGE_CURVE ( 'NONE', #80552, #64315, #79828, .T. ) ;
#113847=AXIS2_PLACEMENT_3D ( 'NONE', #82938, #94033, #71167 ) ;
#113848=AXIS2_PLACEMENT_3D ( 'NONE', #9810, #58913, #98825 ) ;
#113849=ORIENTED_EDGE ( 'NONE', *, *, #98895, .T. ) ;
#113850=DIRECTION ( 'NONE',  ( -0.000000000000000000, 1.000000000000000000, -0.000000000000000000 ) ) ;
#113851=DIRECTION ( 'NONE',  ( -0.000000000000000000, 1.000000000000000000, -0.000000000000000000 ) ) ;
#113852=DIRECTION ( 'NONE',  ( 0.000000000000000000, 0.000000000000000000, 1.000000000000000000 ) ) ;
#113853=ORIENTED_EDGE ( 'NONE', *, *, #120655, .T. ) ;
#113854=ORIENTED_EDGE ( 'NONE', *, *, #52411, .T. ) ;
#113855=CARTESIAN_POINT ( 'NONE',  ( -10.60000000000000320, 2.500000000000000000, -4.576537180435972907 ) ) ;
#113856=EDGE_LOOP ( 'NONE', ( #68550, #79287 ) ) ;
#113857=CARTESIAN_POINT ( 'NONE',  ( -8.100000000000013856, 2.500000000000000000, -3.883716857408426648 ) ) ;
#113858=CARTESIAN_POINT ( 'NONE',  ( -0.8500000000000382805, 2.500000000000000000, -2.857883832488653741 ) ) ;
#113859=CONICAL_SURFACE ( 'NONE', #111811, 0.1000000000000002554, 0.003490658503988666988 ) ;
#113860=VERTEX_POINT ( 'NONE', #41224 ) ;
#113861=AXIS2_PLACEMENT_3D ( 'NONE', #6568, #106730, #36071 ) ;
#113862=CARTESIAN_POINT ( 'NONE',  ( 7.949999999999925571, 2.500000000000000000, -6.595190528383302109 ) ) ;
#113863=LINE ( 'NONE', #64106, #108876 ) ;
#113864=DIRECTION ( 'NONE',  ( 0.000000000000000000, 0.000000000000000000, 1.000000000000000000 ) ) ;
#113865=FACE_OUTER_BOUND ( 'NONE', #120858, .T. ) ;
#113866=DIRECTION ( 'NONE',  ( 0.000000000000000000, 0.000000000000000000, 1.000000000000000000 ) ) ;
#113867=ORIENTED_EDGE ( 'NONE', *, *, #25902, .T. ) ;
#113868=VERTEX_POINT ( 'NONE', #119754 ) ;
#113869=CARTESIAN_POINT ( 'NONE',  ( -6.249999999999984901, 2.500000000000000000, -2.165063509461101710 ) ) ;
#113870=CIRCLE ( 'NONE', #74165, 0.06509327318403745899 ) ;
#113871=CIRCLE ( 'NONE', #94999, 0.1000000000000002554 ) ;
#113873=VERTEX_POINT ( 'NONE', #69355 ) ;
#113874=ORIENTED_EDGE ( 'NONE', *, *, #56633, .F. ) ;
#113875=VERTEX_POINT ( 'NONE', #81136 ) ;
#113876=CIRCLE ( 'NONE', #105268, 0.06509327318403745899 ) ;
#113877=EDGE_CURVE ( 'NONE', #88394, #35493, #69319, .T. ) ;
#113878=DIRECTION ( 'NONE',  ( 0.000000000000000000, 1.000000000000000000, 0.000000000000000000 ) ) ;
#113879=ADVANCED_FACE ( 'NONE', ( #20268 ), #121045, .T. ) ;
#113880=CIRCLE ( 'NONE', #57442, 0.09999999999999982514 ) ;
#113881=DIRECTION ( 'NONE',  ( 0.000000000000000000, 1.000000000000000000, 0.000000000000000000 ) ) ;
#113882=CARTESIAN_POINT ( 'NONE',  ( 4.149999999999941735, 2.500000000000000000, -5.902370205355750521 ) ) ;
#113883=EDGE_CURVE ( 'NONE', #50530, #55864, #44287, .T. ) ;
#113885=DIRECTION ( 'NONE',  ( 0.000000000000000000, 0.000000000000000000, 1.000000000000000000 ) ) ;
#113886=DIRECTION ( 'NONE',  ( 0.000000000000000000, 0.000000000000000000, 1.000000000000000000 ) ) ;
#113888=CARTESIAN_POINT ( 'NONE',  ( -9.999999999999971578, 2.500000000000000000, -4.330127018922197202 ) ) ;
#113889=DIRECTION ( 'NONE',  ( -0.000000000000000000, 1.000000000000000000, -0.000000000000000000 ) ) ;
#113890=EDGE_CURVE ( 'NONE', #57147, #100871, #61504, .T. ) ;
#113891=CARTESIAN_POINT ( 'NONE',  ( 14.14999999999989377, 2.500000000000000000, -1.472243186433550122 ) ) ;
#113892=ADVANCED_FACE ( 'NONE', ( #90274 ), #73526, .T. ) ;
#113893=ADVANCED_FACE ( 'NONE', ( #29453 ), #50372, .T. ) ;
#113894=VERTEX_POINT ( 'NONE', #80497 ) ;
#113895=ADVANCED_FACE ( 'NONE', ( #70656 ), #48409, .T. ) ;
#113896=AXIS2_PLACEMENT_3D ( 'NONE', #59521, #99432, #71234 ) ;
#113897=VECTOR ( 'NONE', #128078, 1000.000000000000000 ) ;
#113898=DIRECTION ( 'NONE',  ( 0.000000000000000000, -0.9999939076577903929, 0.003490651415223739937 ) ) ;
#113899=AXIS2_PLACEMENT_3D ( 'NONE', #19895, #48713, #57889 ) ;
#113900=CIRCLE ( 'NONE', #90905, 0.1000000000000000472 ) ;
#113901=ORIENTED_EDGE ( 'NONE', *, *, #124437, .F. ) ;
#113902=ORIENTED_EDGE ( 'NONE', *, *, #5208, .T. ) ;
#113903=CARTESIAN_POINT ( 'NONE',  ( -14.34999999999998543, 2.500000000000000000, 2.511473670974877503 ) ) ;
#113904=LINE ( 'NONE', #24226, #99063 ) ;
#113905=LINE ( 'NONE', #104700, #123897 ) ;
#113906=EDGE_CURVE ( 'NONE', #15576, #100404, #115275, .T. ) ;
#113908=AXIS2_PLACEMENT_3D ( 'NONE', #102315, #82015, #42771 ) ;
#113909=DIRECTION ( 'NONE',  ( 0.000000000000000000, 1.000000000000000000, 0.000000000000000000 ) ) ;
#113910=CARTESIAN_POINT ( 'NONE',  ( 9.599999999999914380, 2.500000000000000000, 3.637306695894644726 ) ) ;
#113911=DIRECTION ( 'NONE',  ( 0.000000000000000000, 0.000000000000000000, 1.000000000000000000 ) ) ;
#113912=ORIENTED_EDGE ( 'NONE', *, *, #41630, .T. ) ;
#113913=FACE_OUTER_BOUND ( 'NONE', #38096, .T. ) ;
#113914=CIRCLE ( 'NONE', #120263, 0.1000000000000002554 ) ;
#113915=CARTESIAN_POINT ( 'NONE',  ( 6.449999999999931788, 12.50000000000000000, 6.213873640053558134 ) ) ;
#113916=AXIS2_PLACEMENT_3D ( 'NONE', #39073, #8282, #78341 ) ;
#113917=EDGE_LOOP ( 'NONE', ( #129445, #61257 ) ) ;
#113918=VERTEX_POINT ( 'NONE', #5131 ) ;
#113919=VERTEX_POINT ( 'NONE', #103355 ) ;
#113921=VERTEX_POINT ( 'NONE', #105277 ) ;
#113922=CARTESIAN_POINT ( 'NONE',  ( 8.099999999999921485, 2.500000000000000000, -0.2464101615137783419 ) ) ;
#113923=LINE ( 'NONE', #94265, #58221 ) ;
#113924=DIRECTION ( 'NONE',  ( 0.000000000000000000, 0.000000000000000000, 1.000000000000000000 ) ) ;
#113925=CARTESIAN_POINT ( 'NONE',  ( 4.349999999999940137, 2.500000000000000000, -6.941600689897078347 ) ) ;
#113926=CARTESIAN_POINT ( 'NONE',  ( 1.449999999999952216, 12.50000000000000000, 1.883746621131358934 ) ) ;
#113927=ORIENTED_EDGE ( 'NONE', *, *, #19659, .T. ) ;
#113928=CARTESIAN_POINT ( 'NONE',  ( -9.150000000000009237, 12.50000000000000000, -2.857883832488653741 ) ) ;
#113929=DIRECTION ( 'NONE',  ( 0.000000000000000000, 0.000000000000000000, -1.000000000000000000 ) ) ;
#113930=CIRCLE ( 'NONE', #116062, 0.06509327318403745899 ) ;
#113931=DIRECTION ( 'NONE',  ( 0.000000000000000000, 1.000000000000000000, 0.000000000000000000 ) ) ;
#113932=VERTEX_POINT ( 'NONE', #13657 ) ;
#113933=EDGE_CURVE ( 'NONE', #102898, #55074, #75172, .T. ) ;
#113934=VERTEX_POINT ( 'NONE', #94163 ) ;
#113935=VERTEX_POINT ( 'NONE', #115071 ) ;
#113936=CARTESIAN_POINT ( 'NONE',  ( 9.799999999999917222, 12.50000000000000000, 0.4115034346978109769 ) ) ;
#113937=CONICAL_SURFACE ( 'NONE', #19858, 0.1000000000000002554, 0.003490658503988666988 ) ;
#113938=DIRECTION ( 'NONE',  ( 0.000000000000000000, 0.000000000000000000, 1.000000000000000000 ) ) ;
#113940=CIRCLE ( 'NONE', #36590, 0.06509327318403745899 ) ;
#113941=EDGE_LOOP ( 'NONE', ( #35000, #128292 ) ) ;
#113942=DIRECTION ( 'NONE',  ( 0.000000000000000000, -0.9999939076577903929, 0.003490651415223739937 ) ) ;
#113943=CARTESIAN_POINT ( 'NONE',  ( 7.949999999999925571, 2.500000000000000000, 2.165063509461097713 ) ) ;
#113945=DIRECTION ( 'NONE',  ( -0.000000000000000000, 1.000000000000000000, -0.000000000000000000 ) ) ;
#113946=DIRECTION ( 'NONE',  ( 0.000000000000000000, 0.000000000000000000, -1.000000000000000000 ) ) ;
#113947=VECTOR ( 'NONE', #55025, 1000.000000000000000 ) ;
#113948=DIRECTION ( 'NONE',  ( 0.000000000000000000, 0.000000000000000000, -1.000000000000000000 ) ) ;
#113949=CIRCLE ( 'NONE', #57520, 0.09999999999999982514 ) ;
#113950=EDGE_LOOP ( 'NONE', ( #121569, #42452 ) ) ;
#113951=ORIENTED_EDGE ( 'NONE', *, *, #75621, .T. ) ;
#113952=DIRECTION ( 'NONE',  ( -4.274815082592931898E-19, -0.9999939076577903929, -0.003490651415223739937 ) ) ;
#113953=DIRECTION ( 'NONE',  ( 0.000000000000000000, 1.000000000000000000, 0.000000000000000000 ) ) ;
#113954=CARTESIAN_POINT ( 'NONE',  ( 3.149999999999946176, 2.500000000000000000, -1.818653347947325916 ) ) ;
#113955=FACE_OUTER_BOUND ( 'NONE', #61780, .T. ) ;
#113956=DIRECTION ( 'NONE',  ( -0.000000000000000000, -1.000000000000000000, -0.000000000000000000 ) ) ;
#113957=ORIENTED_EDGE ( 'NONE', *, *, #17308, .T. ) ;
#113958=CONICAL_SURFACE ( 'NONE', #53334, 0.09999999999999982514, 0.003490658503988666988 ) ;
#113959=VECTOR ( 'NONE', #31743, 1000.000000000000000 ) ;
#113960=EDGE_LOOP ( 'NONE', ( #58421, #42827 ) ) ;
#113961=CARTESIAN_POINT ( 'NONE',  ( 3.749999999999942268, 2.500000000000000000, 1.472243186433545459 ) ) ;
#113962=DIRECTION ( 'NONE',  ( 0.000000000000000000, -0.9999939076577903929, 0.003490651415223739937 ) ) ;
#113963=CARTESIAN_POINT ( 'NONE',  ( 1.249999999999952038, 12.50000000000000000, -1.472243186433550122 ) ) ;
#113964=CARTESIAN_POINT ( 'NONE',  ( 13.34999999999989662, 2.500000000000000000, -1.572243186433550211 ) ) ;
#113965=EDGE_LOOP ( 'NONE', ( #124202, #121504 ) ) ;
#113966=PLANE ( 'NONE',  #97048 ) ;
#113967=ADVANCED_FACE ( 'NONE', ( #45081 ), #3848, .T. ) ;
#113969=VERTEX_POINT ( 'NONE', #112531 ) ;
#113970=FACE_OUTER_BOUND ( 'NONE', #22896, .T. ) ;
#113971=CIRCLE ( 'NONE', #72226, 0.06509327318403745899 ) ;
#113972=VERTEX_POINT ( 'NONE', #94812 ) ;
#113973=EDGE_CURVE ( 'NONE', #68600, #125596, #121552, .T. ) ;
#113974=CARTESIAN_POINT ( 'NONE',  ( -4.550000000000022915, 2.500000000000000000, 6.595190528383296780 ) ) ;
#113975=CIRCLE ( 'NONE', #111923, 0.06509327318403745899 ) ;
#113976=VERTEX_POINT ( 'NONE', #84980 ) ;
#113977=DIRECTION ( 'NONE',  ( 0.000000000000000000, 0.000000000000000000, 1.000000000000000000 ) ) ;
#113978=FACE_OUTER_BOUND ( 'NONE', #55726, .T. ) ;
#113979=ADVANCED_FACE ( 'NONE', ( #83072 ), #17068, .T. ) ;
#113980=CIRCLE ( 'NONE', #1104, 0.1000000000000000472 ) ;
#113981=ORIENTED_EDGE ( 'NONE', *, *, #27423, .F. ) ;
#113982=ADVANCED_FACE ( 'NONE', ( #63421 ), #31689, .T. ) ;
#113983=ORIENTED_EDGE ( 'NONE', *, *, #72842, .F. ) ;
#113985=EDGE_CURVE ( 'NONE', #65870, #66105, #18174, .T. ) ;
#113987=CARTESIAN_POINT ( 'NONE',  ( 12.89999999999990266, 12.50000000000000000, -3.702399969078687292 ) ) ;
#113989=DIRECTION ( 'NONE',  ( 0.000000000000000000, 1.000000000000000000, 0.000000000000000000 ) ) ;
#113991=CIRCLE ( 'NONE', #91005, 0.1000000000000000472 ) ;
#113992=FACE_OUTER_BOUND ( 'NONE', #47934, .T. ) ;
#113993=DIRECTION ( 'NONE',  ( -0.000000000000000000, 1.000000000000000000, -0.000000000000000000 ) ) ;
#113994=AXIS2_PLACEMENT_3D ( 'NONE', #27160, #36988, #87353 ) ;
#113995=CARTESIAN_POINT ( 'NONE',  ( -3.350000000000031619, 2.500000000000000000, -5.802370205355749988 ) ) ;
#113996=FACE_OUTER_BOUND ( 'NONE', #52364, .T. ) ;
#113997=EDGE_CURVE ( 'NONE', #22231, #119031, #58879, .T. ) ;
#113998=ADVANCED_FACE ( 'NONE', ( #109792 ), #119503, .T. ) ;
#113999=CIRCLE ( 'NONE', #116048, 0.1000000000000002554 ) ;
#114000=CIRCLE ( 'NONE', #86889, 0.06509327318403745899 ) ;
#114001=EDGE_CURVE ( 'NONE', #15869, #23517, #46342, .T. ) ;
#114002=ORIENTED_EDGE ( 'NONE', *, *, #77093, .T. ) ;
#114003=VERTEX_POINT ( 'NONE', #11578 ) ;
#114004=FACE_OUTER_BOUND ( 'NONE', #39160, .T. ) ;
#114005=CARTESIAN_POINT ( 'NONE',  ( 3.749999999999944045, 2.500000000000000000, -7.188010851410854052 ) ) ;
#114006=DIRECTION ( 'NONE',  ( 0.000000000000000000, 1.000000000000000000, 0.000000000000000000 ) ) ;
#114007=AXIS2_PLACEMENT_3D ( 'NONE', #45347, #124549, #52102 ) ;
#114008=DIRECTION ( 'NONE',  ( 0.000000000000000000, 0.000000000000000000, 1.000000000000000000 ) ) ;
#114009=ORIENTED_EDGE ( 'NONE', *, *, #44494, .T. ) ;
#114010=EDGE_LOOP ( 'NONE', ( #11488, #106767, #8074, #64930 ) ) ;
#114011=CARTESIAN_POINT ( 'NONE',  ( 8.149999999999923972, 12.50000000000000000, -6.906693963081115051 ) ) ;
#114012=ORIENTED_EDGE ( 'NONE', *, *, #39816, .T. ) ;
#114013=CARTESIAN_POINT ( 'NONE',  ( 15.59999999999988951, 2.500000000000000000, -0.4464101615137783252 ) ) ;
#114014=CARTESIAN_POINT ( 'NONE',  ( -3.350000000000028955, 2.500000000000000000, 2.165063509461097713 ) ) ;
#114015=EDGE_LOOP ( 'NONE', ( #81735, #77708 ) ) ;
#114016=CARTESIAN_POINT ( 'NONE',  ( -0.4000000000000396572, 12.50000000000000000, 3.637306695894644726 ) ) ;
#114017=DIRECTION ( 'NONE',  ( 0.000000000000000000, -0.000000000000000000, 1.000000000000000000 ) ) ;
#114018=DIRECTION ( 'NONE',  ( -0.000000000000000000, -1.000000000000000000, -0.000000000000000000 ) ) ;
#114019=CARTESIAN_POINT ( 'NONE',  ( 2.499999999999948930, 12.50000000000000000, -0.7579135962115916003 ) ) ;
#114020=CARTESIAN_POINT ( 'NONE',  ( -13.09999999999999254, 12.50000000000000000, -4.676537180435975216 ) ) ;
#114021=DIRECTION ( 'NONE',  ( -0.000000000000000000, -1.000000000000000000, -0.000000000000000000 ) ) ;
#114023=DIRECTION ( 'NONE',  ( 0.000000000000000000, 1.000000000000000000, 0.000000000000000000 ) ) ;
#114024=AXIS2_PLACEMENT_3D ( 'NONE', #30146, #89052, #117841 ) ;
#114025=CARTESIAN_POINT ( 'NONE',  ( -3.350000000000031619, 2.500000000000000000, -5.902370205355750521 ) ) ;
#114026=ORIENTED_EDGE ( 'NONE', *, *, #70107, .F. ) ;
#114027=ORIENTED_EDGE ( 'NONE', *, *, #16324, .F. ) ;
#114028=ORIENTED_EDGE ( 'NONE', *, *, #47660, .F. ) ;
#114029=PLANE ( 'NONE',  #109696 ) ;
#114030=ORIENTED_EDGE ( 'NONE', *, *, #91763, .T. ) ;
#114031=VERTEX_POINT ( 'NONE', #128812 ) ;
#114032=EDGE_LOOP ( 'NONE', ( #2918, #69764 ) ) ;
#114033=EDGE_LOOP ( 'NONE', ( #124601, #123600, #11549, #94041 ) ) ;
#114034=CARTESIAN_POINT ( 'NONE',  ( 0.3999999999999563904, 12.50000000000000000, 5.088040615133786027 ) ) ;
#114035=CONICAL_SURFACE ( 'NONE', #82744, 0.09999999999999982514, 0.003490658503988666988 ) ;
#114036=AXIS2_PLACEMENT_3D ( 'NONE', #17363, #119439, #49448 ) ;
#114037=FACE_OUTER_BOUND ( 'NONE', #116133, .T. ) ;
#114038=DIRECTION ( 'NONE',  ( 0.000000000000000000, 0.000000000000000000, -1.000000000000000000 ) ) ;
#114039=CARTESIAN_POINT ( 'NONE',  ( -1.050000000000037348, 12.50000000000000000, -6.906693963081115939 ) ) ;
#114040=DIRECTION ( 'NONE',  ( -0.000000000000000000, -1.000000000000000000, -0.000000000000000000 ) ) ;
#114041=EDGE_LOOP ( 'NONE', ( #36669, #117049, #18920, #98436 ) ) ;
#114042=EDGE_CURVE ( 'NONE', #44898, #82776, #50651, .T. ) ;
#114043=CARTESIAN_POINT ( 'NONE',  ( 15.39999999999989200, 2.500000000000000000, -0.6928203230275542523 ) ) ;
#114044=ORIENTED_EDGE ( 'NONE', *, *, #41363, .F. ) ;
#114045=VECTOR ( 'NONE', #8489, 1000.000000000000000 ) ;
#114046=EDGE_CURVE ( 'NONE', #25459, #21997, #58973, .T. ) ;
#114047=ORIENTED_EDGE ( 'NONE', *, *, #100123, .T. ) ;
#114048=ORIENTED_EDGE ( 'NONE', *, *, #58717, .T. ) ;
#114049=AXIS2_PLACEMENT_3D ( 'NONE', #82941, #109815, #60086 ) ;
#114050=EDGE_CURVE ( 'NONE', #49778, #110877, #30602, .T. ) ;
#114051=DIRECTION ( 'NONE',  ( -0.000000000000000000, 1.000000000000000000, -0.000000000000000000 ) ) ;
#114052=VERTEX_POINT ( 'NONE', #22068 ) ;
#114053=ORIENTED_EDGE ( 'NONE', *, *, #111124, .T. ) ;
#114054=ORIENTED_EDGE ( 'NONE', *, *, #106888, .T. ) ;
#114055=CARTESIAN_POINT ( 'NONE',  ( -8.550000000000011369, 12.50000000000000000, 1.818653347947321475 ) ) ;
#114056=EDGE_CURVE ( 'NONE', #92222, #54959, #71802, .T. ) ;
#114058=CARTESIAN_POINT ( 'NONE',  ( -6.650000000000018119, 2.500000000000000000, -2.265063509461101798 ) ) ;
#114059=CIRCLE ( 'NONE', #76405, 0.09999999999999982514 ) ;
#114060=CARTESIAN_POINT ( 'NONE',  ( 4.149999999999941735, 2.500000000000000000, -1.372243186433550033 ) ) ;
#114061=FACE_OUTER_BOUND ( 'NONE', #36135, .T. ) ;
#114062=DIRECTION ( 'NONE',  ( 0.000000000000000000, 0.000000000000000000, 1.000000000000000000 ) ) ;
#114063=CARTESIAN_POINT ( 'NONE',  ( 0.5999999999999612310, 2.500000000000000000, -0.3464101615137760715 ) ) ;
#114064=EDGE_LOOP ( 'NONE', ( #119837, #83681 ) ) ;
#114065=DIRECTION ( 'NONE',  ( 0.000000000000000000, 0.000000000000000000, 1.000000000000000000 ) ) ;
#114066=VERTEX_POINT ( 'NONE', #118958 ) ;
#114068=ORIENTED_EDGE ( 'NONE', *, *, #10468, .F. ) ;
#114069=EDGE_CURVE ( 'NONE', #56093, #58995, #88180, .T. ) ;
#114070=EDGE_LOOP ( 'NONE', ( #15093, #45427, #109374, #59851 ) ) ;
#114071=LINE ( 'NONE', #95077, #128533 ) ;
#114073=VECTOR ( 'NONE', #68274, 1000.000000000000000 ) ;
#114074=CARTESIAN_POINT ( 'NONE',  ( -14.39999999999998614, 12.50000000000000000, -0.3464101615137760715 ) ) ;
#114075=ORIENTED_EDGE ( 'NONE', *, *, #38955, .T. ) ;
#114076=DIRECTION ( 'NONE',  ( 0.000000000000000000, 0.000000000000000000, 1.000000000000000000 ) ) ;
#114077=ORIENTED_EDGE ( 'NONE', *, *, #92465, .F. ) ;
#114078=PLANE ( 'NONE',  #18492 ) ;
#114079=CARTESIAN_POINT ( 'NONE',  ( 5.399999999999933742, 2.500000000000000000, -2.385244779468109755E-15 ) ) ;
#114081=CARTESIAN_POINT ( 'NONE',  ( -0.4000000000000392131, 12.50000000000000000, -4.330127018922201643 ) ) ;
#114083=AXIS2_PLACEMENT_3D ( 'NONE', #52399, #104083, #43247 ) ;
#114084=DIRECTION ( 'NONE',  ( 0.000000000000000000, 1.000000000000000000, 0.000000000000000000 ) ) ;
#114085=ORIENTED_EDGE ( 'NONE', *, *, #33624, .T. ) ;
#114086=ADVANCED_FACE ( 'NONE', ( #121520 ), #6693, .T. ) ;
#114087=AXIS2_PLACEMENT_3D ( 'NONE', #48751, #10717, #90587 ) ;
#114088=EDGE_LOOP ( 'NONE', ( #63452, #21190, #98937, #88189 ) ) ;
#114089=AXIS2_PLACEMENT_3D ( 'NONE', #50644, #49379, #89284 ) ;
#114090=FACE_OUTER_BOUND ( 'NONE', #32759, .T. ) ;
#114091=CARTESIAN_POINT ( 'NONE',  ( 10.84999999999991260, 2.500000000000000000, 6.495190528383297135 ) ) ;
#114092=CONICAL_SURFACE ( 'NONE', #80649, 0.09999999999999982514, 0.003490658503988666988 ) ;
#114093=VECTOR ( 'NONE', #59694, 1000.000000000000000 ) ;
#114095=CARTESIAN_POINT ( 'NONE',  ( -5.200000000000022382, 2.500000000000000000, 4.676537180435972552 ) ) ;
#114096=CARTESIAN_POINT ( 'NONE',  ( 2.499999999999945377, 12.50000000000000000, 5.088040615133786027 ) ) ;
#114097=EDGE_CURVE ( 'NONE', #51506, #110134, #19239, .T. ) ;
#114098=CARTESIAN_POINT ( 'NONE',  ( 10.84999999999990905, 2.500000000000000000, 2.265063509461097357 ) ) ;
#114099=CARTESIAN_POINT ( 'NONE',  ( -0.6500000000000394351, 12.50000000000000000, 6.776507416713035248 ) ) ;
#114100=VERTEX_POINT ( 'NONE', #120887 ) ;
#114101=DIRECTION ( 'NONE',  ( 0.000000000000000000, 0.000000000000000000, 1.000000000000000000 ) ) ;
#114102=CARTESIAN_POINT ( 'NONE',  ( -12.09999999999999432, 12.50000000000000000, 5.022947341949748790 ) ) ;
#114104=VERTEX_POINT ( 'NONE', #100597 ) ;
#114105=EDGE_CURVE ( 'NONE', #75943, #100949, #31784, .T. ) ;
#114107=DIRECTION ( 'NONE',  ( -0.000000000000000000, -1.000000000000000000, -0.000000000000000000 ) ) ;
#114109=DIRECTION ( 'NONE',  ( 0.000000000000000000, 0.000000000000000000, 1.000000000000000000 ) ) ;
#114110=CIRCLE ( 'NONE', #82739, 0.06509327318403745899 ) ;
#114111=ORIENTED_EDGE ( 'NONE', *, *, #13944, .T. ) ;
#114112=FACE_OUTER_BOUND ( 'NONE', #112937, .T. ) ;
#114113=CARTESIAN_POINT ( 'NONE',  ( 9.999999999999914735, 12.50000000000000000, 0.6277270498435120194 ) ) ;
#114114=DIRECTION ( 'NONE',  ( -4.274815082592931898E-19, -0.9999939076577903929, -0.003490651415223739937 ) ) ;
#114115=AXIS2_PLACEMENT_3D ( 'NONE', #127822, #118645, #98352 ) ;
#114116=ORIENTED_EDGE ( 'NONE', *, *, #5101, .T. ) ;
#114117=DIRECTION ( 'NONE',  ( -0.000000000000000000, 1.000000000000000000, -0.000000000000000000 ) ) ;
#114118=CIRCLE ( 'NONE', #91133, 0.1000000000000002554 ) ;
#114119=EDGE_CURVE ( 'NONE', #48486, #43713, #104910, .T. ) ;
#114120=DIRECTION ( 'NONE',  ( 0.000000000000000000, -0.000000000000000000, 1.000000000000000000 ) ) ;
#114121=ORIENTED_EDGE ( 'NONE', *, *, #25210, .T. ) ;
#114122=FACE_OUTER_BOUND ( 'NONE', #34069, .T. ) ;
#114123=CIRCLE ( 'NONE', #13860, 0.06509327318403745899 ) ;
#114124=EDGE_CURVE ( 'NONE', #25500, #104198, #54836, .T. ) ;
#114125=ORIENTED_EDGE ( 'NONE', *, *, #121524, .T. ) ;
#114126=VECTOR ( 'NONE', #112591, 1000.000000000000000 ) ;
#114127=AXIS2_PLACEMENT_3D ( 'NONE', #21110, #61037, #37065 ) ;
#114128=VERTEX_POINT ( 'NONE', #129459 ) ;
#114129=CARTESIAN_POINT ( 'NONE',  ( -7.050000000000013145, 2.500000000000000000, 6.495190528383297135 ) ) ;
#114130=CARTESIAN_POINT ( 'NONE',  ( -1.650000000000034328, 12.50000000000000000, -2.922977105672691422 ) ) ;
#114131=DIRECTION ( 'NONE',  ( -0.000000000000000000, 1.000000000000000000, -0.000000000000000000 ) ) ;
#114132=ADVANCED_FACE ( 'NONE', ( #39780 ), #79677, .T. ) ;
#114133=EDGE_CURVE ( 'NONE', #80090, #54834, #23455, .T. ) ;
#114134=ORIENTED_EDGE ( 'NONE', *, *, #4595, .F. ) ;
#114135=ADVANCED_FACE ( 'NONE', ( #1113 ), #41071, .T. ) ;
#114136=ADVANCED_FACE ( 'NONE', ( #61335 ), #41707, .T. ) ;
#114137=DIRECTION ( 'NONE',  ( -0.000000000000000000, 1.000000000000000000, -0.000000000000000000 ) ) ;
#114138=PLANE ( 'NONE',  #92047 ) ;
#114139=ORIENTED_EDGE ( 'NONE', *, *, #9216, .F. ) ;
#114140=CARTESIAN_POINT ( 'NONE',  ( 11.64999999999990443, 2.500000000000000000, -7.088010851410853519 ) ) ;
#114141=DIRECTION ( 'NONE',  ( 0.000000000000000000, 0.000000000000000000, -1.000000000000000000 ) ) ;
#114142=AXIS2_PLACEMENT_3D ( 'NONE', #44628, #64257, #55729 ) ;
#114143=EDGE_CURVE ( 'NONE', #104575, #128976, #94007, .T. ) ;
#114144=CARTESIAN_POINT ( 'NONE',  ( 11.04999999999990656, 2.500000000000000000, -6.248780366869526759 ) ) ;
#114145=CARTESIAN_POINT ( 'NONE',  ( -8.750000000000008882, 12.50000000000000000, -2.792790559304616504 ) ) ;
#114148=LINE ( 'NONE', #24477, #97387 ) ;
#114149=DIRECTION ( 'NONE',  ( 0.000000000000000000, -0.9999939076577903929, 0.003490651415223739937 ) ) ;
#114151=EDGE_CURVE ( 'NONE', #52643, #55268, #8771, .T. ) ;
#114152=ADVANCED_FACE ( 'NONE', ( #82914 ), #115366, .T. ) ;
#114153=VERTEX_POINT ( 'NONE', #94640 ) ;
#114154=VERTEX_POINT ( 'NONE', #34464 ) ;
#114155=ORIENTED_EDGE ( 'NONE', *, *, #53892, .T. ) ;
#114156=ORIENTED_EDGE ( 'NONE', *, *, #34528, .T. ) ;
#114157=CARTESIAN_POINT ( 'NONE',  ( -4.077824815344644402E-14, 2.500000000000000000, -5.122947341949753763 ) ) ;
#114158=CARTESIAN_POINT ( 'NONE',  ( 6.899999999999928413, 2.500000000000000000, 3.883716857408421319 ) ) ;
#114159=DIRECTION ( 'NONE',  ( 0.000000000000000000, 1.000000000000000000, 0.000000000000000000 ) ) ;
#114160=ORIENTED_EDGE ( 'NONE', *, *, #85576, .T. ) ;
#114161=EDGE_CURVE ( 'NONE', #12624, #55645, #107065, .T. ) ;
#114162=FACE_BOUND ( 'NONE', #129569, .T. ) ;
#114163=EDGE_CURVE ( 'NONE', #61624, #69063, #74370, .T. ) ;
#114164=PLANE ( 'NONE',  #14515 ) ;
#114165=PLANE ( 'NONE',  #77211 ) ;
#114166=DIRECTION ( 'NONE',  ( 0.000000000000000000, 0.000000000000000000, 1.000000000000000000 ) ) ;
#114167=AXIS2_PLACEMENT_3D ( 'NONE', #58337, #78624, #98879 ) ;
#114168=CARTESIAN_POINT ( 'NONE',  ( -10.80000000000000071, 12.50000000000000000, 4.330127018922196314 ) ) ;
#114169=AXIS2_PLACEMENT_3D ( 'NONE', #5246, #94931, #85739 ) ;
#114170=DIRECTION ( 'NONE',  ( 0.000000000000000000, -0.9999939076577903929, 0.003490651415223739937 ) ) ;
#114171=DIRECTION ( 'NONE',  ( -0.000000000000000000, -1.000000000000000000, -0.000000000000000000 ) ) ;
#114172=DIRECTION ( 'NONE',  ( 0.000000000000000000, 0.000000000000000000, 1.000000000000000000 ) ) ;
#114173=CARTESIAN_POINT ( 'NONE',  ( -1.250000000000036193, 2.500000000000000000, 1.472243186433545459 ) ) ;
#114174=DIRECTION ( 'NONE',  ( 0.000000000000000000, 0.000000000000000000, 1.000000000000000000 ) ) ;
#114175=CARTESIAN_POINT ( 'NONE',  ( 3.099999999999944134, 2.500000000000000000, 4.576537180435972019 ) ) ;
#114176=AXIS2_PLACEMENT_3D ( 'NONE', #95897, #105721, #124711 ) ;
#114177=CIRCLE ( 'NONE', #57751, 0.06509327318403745899 ) ;
#114178=EDGE_LOOP ( 'NONE', ( #112847, #53786, #53351, #35161 ) ) ;
#114179=EDGE_LOOP ( 'NONE', ( #65253, #127255, #71789, #53563 ) ) ;
#114180=ORIENTED_EDGE ( 'NONE', *, *, #41295, .F. ) ;
#114181=VERTEX_POINT ( 'NONE', #33178 ) ;
#114182=ORIENTED_EDGE ( 'NONE', *, *, #109244, .T. ) ;
#114183=CARTESIAN_POINT ( 'NONE',  ( -11.69999999999999929, 2.500000000000000000, -4.330127018922198978 ) ) ;
#114184=ORIENTED_EDGE ( 'NONE', *, *, #105863, .T. ) ;
#114185=VERTEX_POINT ( 'NONE', #104469 ) ;
#114187=VECTOR ( 'NONE', #124434, 1000.000000000000000 ) ;
#114188=CONICAL_SURFACE ( 'NONE', #64011, 0.1000000000000000056, 0.003490658503988666988 ) ;
#114189=CARTESIAN_POINT ( 'NONE',  ( 13.34999999999990017, 12.50000000000000000, 1.407149913249508000 ) ) ;
#114190=DIRECTION ( 'NONE',  ( 0.000000000000000000, -0.9999939076577903929, 0.003490651415223739937 ) ) ;
#114191=CARTESIAN_POINT ( 'NONE',  ( -4.400000000000025224, 2.500000000000000000, 0.3464101615137735735 ) ) ;
#114192=CARTESIAN_POINT ( 'NONE',  ( -5.450000000000019718, 12.50000000000000000, 2.165063509461097713 ) ) ;
#114193=EDGE_LOOP ( 'NONE', ( #31840, #20106, #58822, #70460 ) ) ;
#114194=EDGE_LOOP ( 'NONE', ( #129308, #7384 ) ) ;
#114195=ADVANCED_FACE ( 'NONE', ( #23988 ), #65202, .T. ) ;
#114196=EDGE_LOOP ( 'NONE', ( #72554, #38231, #104456, #54517 ) ) ;
#114197=DIRECTION ( 'NONE',  ( 0.000000000000000000, 0.000000000000000000, 1.000000000000000000 ) ) ;
#114199=EDGE_CURVE ( 'NONE', #1969, #107840, #83559, .T. ) ;
#114200=DIRECTION ( 'NONE',  ( -4.274815082592931898E-19, -0.9999939076577903929, -0.003490651415223739937 ) ) ;
#114201=ORIENTED_EDGE ( 'NONE', *, *, #69863, .T. ) ;
#114202=CIRCLE ( 'NONE', #70295, 0.09999999999999982514 ) ;
#114203=VERTEX_POINT ( 'NONE', #114290 ) ;
#114204=DIRECTION ( 'NONE',  ( -0.000000000000000000, 1.000000000000000000, -0.000000000000000000 ) ) ;
#114205=EDGE_CURVE ( 'NONE', #29149, #19578, #38129, .T. ) ;
#114206=DIRECTION ( 'NONE',  ( 0.000000000000000000, 1.000000000000000000, 0.000000000000000000 ) ) ;
#114207=DIRECTION ( 'NONE',  ( 0.000000000000000000, 0.000000000000000000, 1.000000000000000000 ) ) ;
#114208=AXIS2_PLACEMENT_3D ( 'NONE', #124689, #54634, #42930 ) ;
#114209=FACE_OUTER_BOUND ( 'NONE', #51837, .T. ) ;
#114210=DIRECTION ( 'NONE',  ( 0.000000000000000000, 1.000000000000000000, 0.000000000000000000 ) ) ;
#114211=CIRCLE ( 'NONE', #74498, 0.09999999999999982514 ) ;
#114212=CONICAL_SURFACE ( 'NONE', #9750, 0.09999999999999982514, 0.003490658503988666988 ) ;
#114213=ADVANCED_FACE ( 'NONE', ( #122194 ), #42251, .T. ) ;
#114214=ORIENTED_EDGE ( 'NONE', *, *, #68001, .F. ) ;
#114216=AXIS2_PLACEMENT_3D ( 'NONE', #89194, #7393, #27056 ) ;
#114217=ORIENTED_EDGE ( 'NONE', *, *, #94645, .F. ) ;
#114218=CARTESIAN_POINT ( 'NONE',  ( 87.50000000000002842, 6.099025433955697295, 4.412011999987998756 ) ) ;
#114219=VERTEX_POINT ( 'NONE', #44921 ) ;
#114220=DIRECTION ( 'NONE',  ( -0.000000000000000000, 1.000000000000000000, -0.000000000000000000 ) ) ;
#114221=CARTESIAN_POINT ( 'NONE',  ( 8.949999999999917577, 2.500000000000000000, -2.411473670974877859 ) ) ;
#114222=DIRECTION ( 'NONE',  ( 0.000000000000000000, 1.000000000000000000, 0.000000000000000000 ) ) ;
#114223=CARTESIAN_POINT ( 'NONE',  ( 8.549999999999922551, 12.50000000000000000, 2.511473670974873507 ) ) ;
#114224=VERTEX_POINT ( 'NONE', #53455 ) ;
#114225=AXIS2_PLACEMENT_3D ( 'NONE', #67587, #118628, #87227 ) ;
#114227=VECTOR ( 'NONE', #104671, 1000.000000000000000 ) ;
#114228=VECTOR ( 'NONE', #124479, 1000.000000000000000 ) ;
#114229=DIRECTION ( 'NONE',  ( 0.000000000000000000, 0.000000000000000000, 1.000000000000000000 ) ) ;
#114230=ORIENTED_EDGE ( 'NONE', *, *, #45358, .F. ) ;
#114231=VERTEX_POINT ( 'NONE', #75020 ) ;
#114232=VERTEX_POINT ( 'NONE', #114924 ) ;
#114233=CARTESIAN_POINT ( 'NONE',  ( 4.199999999999938005, 12.50000000000000000, 4.330127018922196314 ) ) ;
#114234=PLANE ( 'NONE',  #59654 ) ;
#114236=DIRECTION ( 'NONE',  ( -0.000000000000000000, 1.000000000000000000, -0.000000000000000000 ) ) ;
#114237=ADVANCED_FACE ( 'NONE', ( #3692 ), #92402, .T. ) ;
#114238=CARTESIAN_POINT ( 'NONE',  ( 17.45652598566545066, 2.453228361101884580, -4.494719241542722621 ) ) ;
#114239=CARTESIAN_POINT ( 'NONE',  ( -0.4500000000000402012, 2.500000000000000000, 6.495190528383297135 ) ) ;
#114240=VERTEX_POINT ( 'NONE', #25248 ) ;
#114241=FACE_OUTER_BOUND ( 'NONE', #43045, .T. ) ;
#114242=ORIENTED_EDGE ( 'NONE', *, *, #123011, .T. ) ;
#114244=DIRECTION ( 'NONE',  ( 0.000000000000000000, 0.000000000000000000, 1.000000000000000000 ) ) ;
#114245=CARTESIAN_POINT ( 'NONE',  ( -5.200000000000020606, 2.500000000000000000, -0.2464101615137782308 ) ) ;
#114246=CARTESIAN_POINT ( 'NONE',  ( 3.349999999999945466, 2.500000000000000000, -7.288010851410854585 ) ) ;
#114247=VERTEX_POINT ( 'NONE', #32539 ) ;
#114248=CIRCLE ( 'NONE', #22329, 0.06509327318403745899 ) ;
#114249=AXIS2_PLACEMENT_3D ( 'NONE', #47128, #78535, #19591 ) ;
#114250=DIRECTION ( 'NONE',  ( 0.000000000000000000, 0.000000000000000000, 1.000000000000000000 ) ) ;
#114251=DIRECTION ( 'NONE',  ( 0.000000000000000000, 1.000000000000000000, 0.000000000000000000 ) ) ;
#114252=EDGE_CURVE ( 'NONE', #80635, #20888, #113332, .T. ) ;
#114253=ORIENTED_EDGE ( 'NONE', *, *, #10324, .T. ) ;
#114254=VECTOR ( 'NONE', #110077, 1000.000000000000000 ) ;
#114255=CONICAL_SURFACE ( 'NONE', #57841, 0.1000000000000002554, 0.003490658503988666988 ) ;
#114256=DIRECTION ( 'NONE',  ( 0.000000000000000000, 1.000000000000000000, 0.000000000000000000 ) ) ;
#114257=ORIENTED_EDGE ( 'NONE', *, *, #2365, .T. ) ;
#114258=EDGE_LOOP ( 'NONE', ( #119886, #19826, #12809, #98257 ) ) ;
#114259=CARTESIAN_POINT ( 'NONE',  ( 6.249999999999930722, 2.500000000000000000, 7.288010851410849256 ) ) ;
#114260=ORIENTED_EDGE ( 'NONE', *, *, #75437, .T. ) ;
#114261=CARTESIAN_POINT ( 'NONE',  ( 16.79927703354236357, 2.472530191752521311, -3.248144252803072618 ) ) ;
#114262=PLANE ( 'NONE',  #119552 ) ;
#114263=CONICAL_SURFACE ( 'NONE', #74558, 0.1000000000000002554, 0.003490658503988666988 ) ;
#114264=DIRECTION ( 'NONE',  ( 0.000000000000000000, 0.000000000000000000, 1.000000000000000000 ) ) ;
#114265=VERTEX_POINT ( 'NONE', #73711 ) ;
#114266=CONICAL_SURFACE ( 'NONE', #68201, 0.1000000000000002554, 0.003490658503988666988 ) ;
#114267=DIRECTION ( 'NONE',  ( 0.000000000000000000, 1.000000000000000000, 0.000000000000000000 ) ) ;
#114268=LINE ( 'NONE', #27178, #16528 ) ;
#114269=EDGE_LOOP ( 'NONE', ( #89582, #32668, #104131, #72569 ) ) ;
#114270=LINE ( 'NONE', #64523, #117561 ) ;
#114271=DIRECTION ( 'NONE',  ( -0.000000000000000000, -1.000000000000000000, -0.000000000000000000 ) ) ;
#114272=ORIENTED_EDGE ( 'NONE', *, *, #56174, .F. ) ;
#114273=EDGE_CURVE ( 'NONE', #108629, #13143, #100804, .T. ) ;
#114274=ORIENTED_EDGE ( 'NONE', *, *, #114881, .T. ) ;
#114275=EDGE_LOOP ( 'NONE', ( #8005, #106523 ) ) ;
#114276=LINE ( 'NONE', #16057, #104703 ) ;
#114277=PLANE ( 'NONE',  #118921 ) ;
#114278=CARTESIAN_POINT ( 'NONE',  ( 5.649999999999932854, 12.50000000000000000, 2.511473670974873507 ) ) ;
#114279=EDGE_CURVE ( 'NONE', #88674, #117051, #35984, .T. ) ;
#114280=FACE_BOUND ( 'NONE', #101187, .T. ) ;
#114281=EDGE_LOOP ( 'NONE', ( #12836, #95776, #56463, #28488 ) ) ;
#114282=CONICAL_SURFACE ( 'NONE', #39098, 0.1000000000000002554, 0.003490658503988666988 ) ;
#114284=EDGE_CURVE ( 'NONE', #7581, #109083, #115561, .T. ) ;
#114285=DIRECTION ( 'NONE',  ( 0.000000000000000000, -0.000000000000000000, 1.000000000000000000 ) ) ;
#114286=DIRECTION ( 'NONE',  ( 0.000000000000000000, 0.000000000000000000, 1.000000000000000000 ) ) ;
#114287=VECTOR ( 'NONE', #97105, 1000.000000000000000 ) ;
#114288=DIRECTION ( 'NONE',  ( 0.000000000000000000, 0.000000000000000000, 1.000000000000000000 ) ) ;
#114289=ADVANCED_FACE ( 'NONE', ( #126701 ), #117510, .T. ) ;
#114290=CARTESIAN_POINT ( 'NONE',  ( -0.8500000000000386136, 12.50000000000000000, 7.253104124594885960 ) ) ;
#114291=ADVANCED_FACE ( 'NONE', ( #76310 ), #10904, .T. ) ;
#114292=DIRECTION ( 'NONE',  ( 0.000000000000000000, -0.000000000000000000, 1.000000000000000000 ) ) ;
#114293=ADVANCED_FACE ( 'NONE', ( #117483 ), #34018, .T. ) ;
#114294=DIRECTION ( 'NONE',  ( 0.000000000000000000, 0.000000000000000000, 1.000000000000000000 ) ) ;
#114295=AXIS2_PLACEMENT_3D ( 'NONE', #37840, #127519, #4646 ) ;
#114296=DIRECTION ( 'NONE',  ( 0.000000000000000000, 0.000000000000000000, 1.000000000000000000 ) ) ;
#114297=AXIS2_PLACEMENT_3D ( 'NONE', #60350, #111337, #100262 ) ;
#114298=EDGE_CURVE ( 'NONE', #100751, #84404, #5607, .T. ) ;
#114299=ORIENTED_EDGE ( 'NONE', *, *, #97027, .T. ) ;
#114301=EDGE_LOOP ( 'NONE', ( #98980, #41342, #64678, #117891 ) ) ;
#114302=ORIENTED_EDGE ( 'NONE', *, *, #113877, .F. ) ;
#114303=EDGE_LOOP ( 'NONE', ( #121345, #55741, #39048, #75090 ) ) ;
#114304=CARTESIAN_POINT ( 'NONE',  ( 6.449999999999930012, 2.500000000000000000, 6.941600689897073018 ) ) ;
#114305=CARTESIAN_POINT ( 'NONE',  ( 5.799999999999933209, 2.500000000000000000, 0.09999999999999761857 ) ) ;
#114307=ORIENTED_EDGE ( 'NONE', *, *, #46154, .F. ) ;
#114308=FACE_BOUND ( 'NONE', #104572, .T. ) ;
#114309=EDGE_CURVE ( 'NONE', #102404, #105289, #38235, .T. ) ;
#114310=AXIS2_PLACEMENT_3D ( 'NONE', #94984, #64223, #5292 ) ;
#114311=DIRECTION ( 'NONE',  ( 0.000000000000000000, -0.000000000000000000, 1.000000000000000000 ) ) ;
#114312=AXIS2_PLACEMENT_3D ( 'NONE', #90696, #80889, #41621 ) ;
#114313=VECTOR ( 'NONE', #128355, 1000.000000000000000 ) ;
#114314=CARTESIAN_POINT ( 'NONE',  ( 6.049999999999932321, 2.500000000000000000, 6.841600689897072485 ) ) ;
#114315=VERTEX_POINT ( 'NONE', #105105 ) ;
#114316=DIRECTION ( 'NONE',  ( -4.274815082592931898E-19, -0.9999939076577903929, -0.003490651415223739937 ) ) ;
#114317=CARTESIAN_POINT ( 'NONE',  ( -13.74999999999998757, 2.500000000000000000, -2.957883832488651610 ) ) ;
#114318=CARTESIAN_POINT ( 'NONE',  ( -6.450000000000017941, 12.50000000000000000, -6.776507416713039689 ) ) ;
#114319=EDGE_LOOP ( 'NONE', ( #40816, #41543 ) ) ;
#114320=DIRECTION ( 'NONE',  ( 0.000000000000000000, -0.000000000000000000, 1.000000000000000000 ) ) ;
#114321=ORIENTED_EDGE ( 'NONE', *, *, #44394, .F. ) ;
#114322=VERTEX_POINT ( 'NONE', #57314 ) ;
#114323=VERTEX_POINT ( 'NONE', #67769 ) ;
#114324=DIRECTION ( 'NONE',  ( -0.000000000000000000, -1.000000000000000000, -0.000000000000000000 ) ) ;
#114325=CARTESIAN_POINT ( 'NONE',  ( 3.549999999999941203, 12.50000000000000000, 6.148780366869520897 ) ) ;
#114326=CARTESIAN_POINT ( 'NONE',  ( 14.14999999999989377, 2.500000000000000000, -1.372243186433550033 ) ) ;
#114327=ORIENTED_EDGE ( 'NONE', *, *, #115408, .T. ) ;
#114328=CARTESIAN_POINT ( 'NONE',  ( -9.150000000000009237, 12.50000000000000000, -2.165063509461101710 ) ) ;
#114329=CARTESIAN_POINT ( 'NONE',  ( 0.8499999999999527933, 12.50000000000000000, 7.188010851410848723 ) ) ;
#114330=DIRECTION ( 'NONE',  ( 0.000000000000000000, 0.000000000000000000, 1.000000000000000000 ) ) ;
#114331=FACE_OUTER_BOUND ( 'NONE', #27586, .T. ) ;
#114332=CARTESIAN_POINT ( 'NONE',  ( 1.249999999999953815, 2.500000000000000000, -2.857883832488653741 ) ) ;
#114333=EDGE_LOOP ( 'NONE', ( #69121, #127632 ) ) ;
#114334=DIRECTION ( 'NONE',  ( 0.000000000000000000, 1.000000000000000000, 0.000000000000000000 ) ) ;
#114335=EDGE_LOOP ( 'NONE', ( #124095, #28547, #77403, #18544 ) ) ;
#114336=DIRECTION ( 'NONE',  ( 0.000000000000000000, 1.000000000000000000, 0.000000000000000000 ) ) ;
#114337=ORIENTED_EDGE ( 'NONE', *, *, #14407, .F. ) ;
#114338=EDGE_CURVE ( 'NONE', #2220, #41822, #25921, .T. ) ;
#114339=ORIENTED_EDGE ( 'NONE', *, *, #81555, .T. ) ;
#114340=CARTESIAN_POINT ( 'NONE',  ( 5.649999999999934630, 12.50000000000000000, 6.841600689897072485 ) ) ;
#114341=CARTESIAN_POINT ( 'NONE',  ( 2.099999999999949463, 2.500000000000000000, 0.6928203230275494784 ) ) ;
#114342=CARTESIAN_POINT ( 'NONE',  ( 12.09999999999990550, 2.500000000000000000, 3.637306695894644726 ) ) ;
#114343=DIRECTION ( 'NONE',  ( 0.000000000000000000, 1.000000000000000000, 0.000000000000000000 ) ) ;
#114344=CARTESIAN_POINT ( 'NONE',  ( -7.100000000000018296, 2.500000000000000000, -2.385244779468109755E-15 ) ) ;
#114345=EDGE_LOOP ( 'NONE', ( #50912, #81352, #87951, #63208 ) ) ;
#114346=CIRCLE ( 'NONE', #7729, 0.09999999999999982514 ) ;
#114347=AXIS2_PLACEMENT_3D ( 'NONE', #102857, #31565, #102241 ) ;
#114348=EDGE_LOOP ( 'NONE', ( #26358, #74345, #81218, #33808 ) ) ;
#114349=ADVANCED_FACE ( 'NONE', ( #126035 ), #116214, .T. ) ;
#114350=CARTESIAN_POINT ( 'NONE',  ( 10.79999999999991012, 12.50000000000000000, -4.330127018922201643 ) ) ;
#114351=DIRECTION ( 'NONE',  ( 0.000000000000000000, 0.000000000000000000, 1.000000000000000000 ) ) ;
#114352=DIRECTION ( 'NONE',  ( 0.000000000000000000, 0.000000000000000000, 1.000000000000000000 ) ) ;
#114353=ORIENTED_EDGE ( 'NONE', *, *, #44883, .F. ) ;
#114354=ORIENTED_EDGE ( 'NONE', *, *, #49296, .F. ) ;
#114355=CARTESIAN_POINT ( 'NONE',  ( 10.59999999999991260, 2.500000000000000000, -0.4464101615137783252 ) ) ;
#114356=VECTOR ( 'NONE', #66147, 1000.000000000000000 ) ;
#114357=EDGE_LOOP ( 'NONE', ( #121703, #20314, #103756, #125623 ) ) ;
#114358=DIRECTION ( 'NONE',  ( 0.000000000000000000, 0.000000000000000000, -1.000000000000000000 ) ) ;
#114359=CONICAL_SURFACE ( 'NONE', #74649, 0.1000000000000002554, 0.003490658503988666988 ) ;
#114360=DIRECTION ( 'NONE',  ( 0.000000000000000000, -0.000000000000000000, 1.000000000000000000 ) ) ;
#114361=EDGE_LOOP ( 'NONE', ( #96970, #58207, #114781, #24885 ) ) ;
#114362=CARTESIAN_POINT ( 'NONE',  ( 7.299999999999927880, 2.500000000000000000, 4.083716857408421497 ) ) ;
#114363=DIRECTION ( 'NONE',  ( -0.000000000000000000, -1.000000000000000000, -0.000000000000000000 ) ) ;
#114364=CARTESIAN_POINT ( 'NONE',  ( 15.39999999999989022, 2.500000000000000000, -2.385244779468109755E-15 ) ) ;
#114365=DIRECTION ( 'NONE',  ( 0.000000000000000000, 1.000000000000000000, 0.000000000000000000 ) ) ;
#114366=ORIENTED_EDGE ( 'NONE', *, *, #78837, .T. ) ;
#114367=DIRECTION ( 'NONE',  ( 0.000000000000000000, 0.000000000000000000, 1.000000000000000000 ) ) ;
#114368=CARTESIAN_POINT ( 'NONE',  ( 81.97620568556726539, -3.937821662896079378, 6.124242991616513976 ) ) ;
#114369=ORIENTED_EDGE ( 'NONE', *, *, #115850, .F. ) ;
#114370=ORIENTED_EDGE ( 'NONE', *, *, #98418, .T. ) ;
#114372=DIRECTION ( 'NONE',  ( 0.000000000000000000, 0.000000000000000000, -1.000000000000000000 ) ) ;
#114373=CARTESIAN_POINT ( 'NONE',  ( 6.849999999999929479, 12.50000000000000000, -2.511473670974877948 ) ) ;
#114374=AXIS2_PLACEMENT_3D ( 'NONE', #103398, #31441, #53645 ) ;
#114376=CARTESIAN_POINT ( 'NONE',  ( -5.650000000000023448, 2.500000000000000000, -1.918653347947326004 ) ) ;
#114377=ADVANCED_FACE ( 'NONE', ( #7549 ), #87396, .T. ) ;
#114378=DIRECTION ( 'NONE',  ( 0.000000000000000000, 0.000000000000000000, 1.000000000000000000 ) ) ;
#114379=CARTESIAN_POINT ( 'NONE',  ( 10.64999999999990976, 2.500000000000000000, 2.511473670974873507 ) ) ;
#114380=CARTESIAN_POINT ( 'NONE',  ( -4.350000000000023626, 12.50000000000000000, 6.213873640053559022 ) ) ;
#114381=DIRECTION ( 'NONE',  ( 0.000000000000000000, 0.000000000000000000, 1.000000000000000000 ) ) ;
#114382=AXIS2_PLACEMENT_3D ( 'NONE', #20642, #60578, #128685 ) ;
#114383=FACE_OUTER_BOUND ( 'NONE', #32986, .T. ) ;
#114384=ADVANCED_FACE ( 'NONE', ( #116858 ), #119686, .T. ) ;
#114385=VERTEX_POINT ( 'NONE', #95943 ) ;
#114386=VERTEX_POINT ( 'NONE', #106403 ) ;
#114387=CIRCLE ( 'NONE', #64215, 0.1000000000000000472 ) ;
#114389=EDGE_CURVE ( 'NONE', #11701, #55594, #65827, .T. ) ;
#114390=VERTEX_POINT ( 'NONE', #37031 ) ;
#114391=CONICAL_SURFACE ( 'NONE', #18253, 0.1000000000000002554, 0.003490658503988666988 ) ;
#114392=CARTESIAN_POINT ( 'NONE',  ( 15.39999999999989022, 12.50000000000000000, -2.385244779468109755E-15 ) ) ;
#114393=EDGE_CURVE ( 'NONE', #79899, #114770, #127351, .T. ) ;
#114394=DIRECTION ( 'NONE',  ( 0.000000000000000000, 0.000000000000000000, 1.000000000000000000 ) ) ;
#114395=LINE ( 'NONE', #14877, #58401 ) ;
#114396=EDGE_LOOP ( 'NONE', ( #60788, #43435 ) ) ;
#114397=FACE_OUTER_BOUND ( 'NONE', #54596, .T. ) ;
#114398=CIRCLE ( 'NONE', #57982, 0.1000000000000000472 ) ;
#114399=CIRCLE ( 'NONE', #118606, 0.06509327318403745899 ) ;
#114400=ADVANCED_FACE ( 'NONE', ( #77576 ), #31873, .T. ) ;
#114401=CARTESIAN_POINT ( 'NONE',  ( 2.699999999999946443, 12.50000000000000000, -3.983716857408426293 ) ) ;
#114402=DIRECTION ( 'NONE',  ( 0.000000000000000000, 1.000000000000000000, 0.000000000000000000 ) ) ;
#114403=VERTEX_POINT ( 'NONE', #48141 ) ;
#114404=EDGE_CURVE ( 'NONE', #104514, #127159, #111353, .T. ) ;
#114405=FACE_OUTER_BOUND ( 'NONE', #109142, .T. ) ;
#114406=CARTESIAN_POINT ( 'NONE',  ( 11.84999999999990372, 2.500000000000000000, 2.511473670974873507 ) ) ;
#114407=ORIENTED_EDGE ( 'NONE', *, *, #5193, .T. ) ;
#114408=ORIENTED_EDGE ( 'NONE', *, *, #83348, .F. ) ;
#114409=EDGE_LOOP ( 'NONE', ( #14110, #110157, #13604, #20672 ) ) ;
#114410=ORIENTED_EDGE ( 'NONE', *, *, #40074, .T. ) ;
#114412=AXIS2_PLACEMENT_3D ( 'NONE', #109013, #79579, #78945 ) ;
#114413=LINE ( 'NONE', #34599, #59302 ) ;
#114414=CARTESIAN_POINT ( 'NONE',  ( 0.3999999999999619971, 2.500000000000000000, -1.084202172485504434E-16 ) ) ;
#114416=ORIENTED_EDGE ( 'NONE', *, *, #90134, .F. ) ;
#114417=EDGE_CURVE ( 'NONE', #23243, #52693, #15208, .T. ) ;
#114418=FACE_OUTER_BOUND ( 'NONE', #67906, .T. ) ;
#114419=EDGE_LOOP ( 'NONE', ( #74386, #79078, #121454, #28636 ) ) ;
#114420=DIRECTION ( 'NONE',  ( -0.000000000000000000, 1.000000000000000000, -0.000000000000000000 ) ) ;
#114421=CARTESIAN_POINT ( 'NONE',  ( 2.499999999999948930, 2.500000000000000000, -0.6928203230275541413 ) ) ;
#114422=DIRECTION ( 'NONE',  ( 0.000000000000000000, 1.000000000000000000, 0.000000000000000000 ) ) ;
#114423=DIRECTION ( 'NONE',  ( 0.000000000000000000, -0.9999939076577903929, 0.003490651415223739937 ) ) ;
#114424=ORIENTED_EDGE ( 'NONE', *, *, #125825, .T. ) ;
#114425=AXIS2_PLACEMENT_3D ( 'NONE', #30347, #127247, #59154 ) ;
#114426=EDGE_CURVE ( 'NONE', #13310, #129065, #123888, .T. ) ;
#114427=VERTEX_POINT ( 'NONE', #51377 ) ;
#114428=ORIENTED_EDGE ( 'NONE', *, *, #62279, .F. ) ;
#114429=CARTESIAN_POINT ( 'NONE',  ( -0.2000000000000404232, 2.500000000000000000, 3.883716857408421319 ) ) ;
#114430=DIRECTION ( 'NONE',  ( -0.000000000000000000, -1.000000000000000000, -0.000000000000000000 ) ) ;
#114431=DIRECTION ( 'NONE',  ( -0.000000000000000000, 1.000000000000000000, -0.000000000000000000 ) ) ;
#114432=FACE_BOUND ( 'NONE', #16761, .T. ) ;
#114433=DIRECTION ( 'NONE',  ( 0.000000000000000000, 0.000000000000000000, 1.000000000000000000 ) ) ;
#114434=FACE_OUTER_BOUND ( 'NONE', #103030, .T. ) ;
#114435=CIRCLE ( 'NONE', #58023, 0.1000000000000002554 ) ;
#114436=CIRCLE ( 'NONE', #81000, 0.1000000000000000472 ) ;
#114437=ADVANCED_FACE ( 'NONE', ( #961 ), #105011, .T. ) ;
#114438=DIRECTION ( 'NONE',  ( 0.000000000000000000, 0.000000000000000000, -1.000000000000000000 ) ) ;
#114439=VECTOR ( 'NONE', #34200, 1000.000000000000000 ) ;
#114440=ADVANCED_FACE ( 'NONE', ( #128661 ), #40286, .T. ) ;
#114442=CARTESIAN_POINT ( 'NONE',  ( -10.65000000000000213, 12.50000000000000000, 2.511473670974873507 ) ) ;
#114443=ADVANCED_FACE ( 'NONE', ( #91279 ), #113437, .T. ) ;
#114444=DIRECTION ( 'NONE',  ( 1.000000000000000000, 0.000000000000000000, 0.000000000000000000 ) ) ;
#114445=EDGE_LOOP ( 'NONE', ( #84131, #72148 ) ) ;
#114446=CONICAL_SURFACE ( 'NONE', #126979, 0.1000000000000002554, 0.003490658503988666988 ) ;
#114447=EDGE_CURVE ( 'NONE', #41701, #35924, #40257, .T. ) ;
#114448=CIRCLE ( 'NONE', #110251, 0.06509327318403745899 ) ;
#114449=DIRECTION ( 'NONE',  ( -0.000000000000000000, -1.000000000000000000, -0.000000000000000000 ) ) ;
#114450=EDGE_CURVE ( 'NONE', #34926, #120592, #20614, .T. ) ;
#114451=EDGE_LOOP ( 'NONE', ( #9995, #13472, #4422, #20053 ) ) ;
#114452=EDGE_LOOP ( 'NONE', ( #109379, #110431 ) ) ;
#114453=ORIENTED_EDGE ( 'NONE', *, *, #114273, .T. ) ;
#114454=VERTEX_POINT ( 'NONE', #39635 ) ;
#114455=CARTESIAN_POINT ( 'NONE',  ( -8.150000000000012790, 12.50000000000000000, 1.818653347947321475 ) ) ;
#114456=FACE_BOUND ( 'NONE', #2374, .T. ) ;
#114457=CARTESIAN_POINT ( 'NONE',  ( -13.29999999999999005, 2.500000000000000000, -0.09999999999999815981 ) ) ;
#114458=ADVANCED_FACE ( 'NONE', ( #8836 ), #50746, .T. ) ;
#114459=AXIS2_PLACEMENT_3D ( 'NONE', #9315, #49260, #81912 ) ;
#114460=EDGE_CURVE ( 'NONE', #73591, #107817, #65297, .T. ) ;
#114461=AXIS2_PLACEMENT_3D ( 'NONE', #67454, #9206, #87754 ) ;
#114462=VERTEX_POINT ( 'NONE', #69054 ) ;
#114464=CARTESIAN_POINT ( 'NONE',  ( 65.40763333621140418, 3.109051995140788005, 5.794606894440900824 ) ) ;
#114465=DIRECTION ( 'NONE',  ( 0.000000000000000000, -0.9999939076577903929, 0.003490651415223739937 ) ) ;
#114466=CIRCLE ( 'NONE', #9923, 0.06509327318403745899 ) ;
#114467=VERTEX_POINT ( 'NONE', #69707 ) ;
#114468=CARTESIAN_POINT ( 'NONE',  ( 2.499999999999947153, 2.500000000000000000, 0.7928203230275495672 ) ) ;
#114469=CONICAL_SURFACE ( 'NONE', #45530, 0.1000000000000000472, 0.003490658503988666988 ) ;
#114470=CARTESIAN_POINT ( 'NONE',  ( -14.34999999999998543, 2.500000000000000000, -1.718653347947323606 ) ) ;
#114472=EDGE_LOOP ( 'NONE', ( #91132, #118493, #110671, #110982 ) ) ;
#114473=DIRECTION ( 'NONE',  ( 0.000000000000000000, 0.000000000000000000, 1.000000000000000000 ) ) ;
#114474=FACE_OUTER_BOUND ( 'NONE', #112444, .T. ) ;
#114475=CIRCLE ( 'NONE', #16253, 0.06509327318403745899 ) ;
#114476=AXIS2_PLACEMENT_3D ( 'NONE', #89380, #57990, #97892 ) ;
#114477=ORIENTED_EDGE ( 'NONE', *, *, #16430, .T. ) ;
#114478=CIRCLE ( 'NONE', #49761, 0.06509327318403741736 ) ;
#114479=FACE_OUTER_BOUND ( 'NONE', #124714, .T. ) ;
#114481=CARTESIAN_POINT ( 'NONE',  ( -7.100000000000013856, 2.500000000000000000, 5.122947341949749323 ) ) ;
#114482=VERTEX_POINT ( 'NONE', #120104 ) ;
#114483=EDGE_LOOP ( 'NONE', ( #100028, #119067, #33718, #55721 ) ) ;
#114484=AXIS2_PLACEMENT_3D ( 'NONE', #106464, #118220, #58026 ) ;
#114485=CARTESIAN_POINT ( 'NONE',  ( -6.250000000000017764, 2.500000000000000000, 7.188010851410848723 ) ) ;
#114486=ORIENTED_EDGE ( 'NONE', *, *, #3079, .F. ) ;
#114487=DIRECTION ( 'NONE',  ( 0.000000000000000000, 0.000000000000000000, 1.000000000000000000 ) ) ;
#114488=CARTESIAN_POINT ( 'NONE',  ( -6.650000000000015454, 12.50000000000000000, 7.188010851410848723 ) ) ;
#114489=AXIS2_PLACEMENT_3D ( 'NONE', #20010, #109004, #8868 ) ;
#114490=EDGE_LOOP ( 'NONE', ( #93741, #126867, #89060, #7745 ) ) ;
#114491=CARTESIAN_POINT ( 'NONE',  ( 1.849999999999950129, 2.500000000000000000, -6.841600689897078702 ) ) ;
#114492=DIRECTION ( 'NONE',  ( 0.000000000000000000, -0.9999939076577903929, 0.003490651415223739937 ) ) ;
#114493=DIRECTION ( 'NONE',  ( 0.000000000000000000, -0.9999939076577903929, 0.003490651415223739937 ) ) ;
#114494=DIRECTION ( 'NONE',  ( -4.274815082592931898E-19, -0.9999939076577903929, -0.003490651415223739937 ) ) ;
#114495=CARTESIAN_POINT ( 'NONE',  ( -2.900000000000029665, 2.500000000000000000, 4.330127018922196314 ) ) ;
#114496=ORIENTED_EDGE ( 'NONE', *, *, #99979, .T. ) ;
#114497=EDGE_CURVE ( 'NONE', #33480, #45085, #56979, .T. ) ;
#114498=ORIENTED_EDGE ( 'NONE', *, *, #45455, .T. ) ;
#114499=DIRECTION ( 'NONE',  ( 0.000000000000000000, -0.000000000000000000, 1.000000000000000000 ) ) ;
#114500=DIRECTION ( 'NONE',  ( 0.000000000000000000, 1.000000000000000000, 0.000000000000000000 ) ) ;
#114501=DIRECTION ( 'NONE',  ( 0.000000000000000000, 0.000000000000000000, -1.000000000000000000 ) ) ;
#114502=ORIENTED_EDGE ( 'NONE', *, *, #113153, .F. ) ;
#114503=ORIENTED_EDGE ( 'NONE', *, *, #59049, .T. ) ;
#114504=EDGE_LOOP ( 'NONE', ( #122388, #59924 ) ) ;
#114505=CARTESIAN_POINT ( 'NONE',  ( 3.349999999999943689, 2.500000000000000000, 1.472243186433545459 ) ) ;
#114506=DIRECTION ( 'NONE',  ( -0.000000000000000000, 1.000000000000000000, -0.000000000000000000 ) ) ;
#114507=LINE ( 'NONE', #7126, #83188 ) ;
#114509=LINE ( 'NONE', #2617, #66146 ) ;
#114510=DIRECTION ( 'NONE',  ( 0.000000000000000000, 0.000000000000000000, -1.000000000000000000 ) ) ;
#114512=PLANE ( 'NONE',  #107716 ) ;
#114513=CARTESIAN_POINT ( 'NONE',  ( 3.549999999999943867, 2.500000000000000000, -1.818653347947326138 ) ) ;
#114514=CARTESIAN_POINT ( 'NONE',  ( 7.049999999999926992, 12.50000000000000000, 2.230156782645134950 ) ) ;
#114515=EDGE_LOOP ( 'NONE', ( #36487, #12279 ) ) ;
#114516=CONICAL_SURFACE ( 'NONE', #14161, 0.1000000000000002554, 0.003490658503988666988 ) ;
#114517=CARTESIAN_POINT ( 'NONE',  ( 2.899999999999946620, 2.500000000000000000, -4.922947341949753586 ) ) ;
#114518=ORIENTED_EDGE ( 'NONE', *, *, #89517, .T. ) ;
#114519=ORIENTED_EDGE ( 'NONE', *, *, #67657, .F. ) ;
#114520=FACE_OUTER_BOUND ( 'NONE', #62659, .T. ) ;
#114521=DIRECTION ( 'NONE',  ( -4.274815082592931898E-19, -0.9999939076577903929, -0.003490651415223739937 ) ) ;
#114522=DIRECTION ( 'NONE',  ( -0.000000000000000000, -1.000000000000000000, -0.000000000000000000 ) ) ;
#114523=CIRCLE ( 'NONE', #1657, 0.09999999999999982514 ) ;
#114524=DIRECTION ( 'NONE',  ( 0.000000000000000000, 0.000000000000000000, 1.000000000000000000 ) ) ;
#114525=VECTOR ( 'NONE', #49188, 1000.000000000000000 ) ;
#114526=AXIS2_PLACEMENT_3D ( 'NONE', #103343, #13648, #101407 ) ;
#114527=DIRECTION ( 'NONE',  ( 0.000000000000000000, 0.000000000000000000, -1.000000000000000000 ) ) ;
#114528=CARTESIAN_POINT ( 'NONE',  ( 9.399999999999918643, 12.50000000000000000, 0.4115034346978110880 ) ) ;
#114529=DIRECTION ( 'NONE',  ( 0.000000000000000000, 0.000000000000000000, 1.000000000000000000 ) ) ;
#114530=ORIENTED_EDGE ( 'NONE', *, *, #107886, .T. ) ;
#114531=DIRECTION ( 'NONE',  ( 0.000000000000000000, 0.000000000000000000, 1.000000000000000000 ) ) ;
#114532=CARTESIAN_POINT ( 'NONE',  ( -4.150000000000025224, 12.50000000000000000, 7.122917578226811486 ) ) ;
#114533=ORIENTED_EDGE ( 'NONE', *, *, #32738, .T. ) ;
#114534=CIRCLE ( 'NONE', #104089, 0.1000000000000002554 ) ;
#114535=ADVANCED_FACE ( 'NONE', ( #81469 ), #102966, .T. ) ;
#114536=EDGE_LOOP ( 'NONE', ( #25605, #125589 ) ) ;
#114537=ORIENTED_EDGE ( 'NONE', *, *, #50306, .F. ) ;
#114538=EDGE_CURVE ( 'NONE', #49438, #65903, #59265, .T. ) ;
#114539=VERTEX_POINT ( 'NONE', #99176 ) ;
#114540=EDGE_CURVE ( 'NONE', #110245, #94388, #90632, .T. ) ;
#114541=DIRECTION ( 'NONE',  ( 0.000000000000000000, 0.000000000000000000, 1.000000000000000000 ) ) ;
#114542=FACE_OUTER_BOUND ( 'NONE', #56149, .T. ) ;
#114543=CIRCLE ( 'NONE', #85302, 0.06509327318403745899 ) ;
#114544=DIRECTION ( 'NONE',  ( 0.000000000000000000, 1.000000000000000000, 0.000000000000000000 ) ) ;
#114545=DIRECTION ( 'NONE',  ( 0.000000000000000000, 0.000000000000000000, 1.000000000000000000 ) ) ;
#114546=EDGE_CURVE ( 'NONE', #10471, #76809, #68408, .T. ) ;
#114547=CARTESIAN_POINT ( 'NONE',  ( -8.750000000000008882, 2.500000000000000000, 1.472243186433545459 ) ) ;
#114548=EDGE_CURVE ( 'NONE', #83056, #9531, #129300, .T. ) ;
#114549=ORIENTED_EDGE ( 'NONE', *, *, #62469, .F. ) ;
#114550=CARTESIAN_POINT ( 'NONE',  ( 3.749999999999944045, 2.500000000000000000, -7.088010851410853519 ) ) ;
#114551=EDGE_CURVE ( 'NONE', #18098, #37160, #17258, .T. ) ;
#114552=EDGE_CURVE ( 'NONE', #64139, #14119, #13058, .T. ) ;
#114553=DIRECTION ( 'NONE',  ( 0.000000000000000000, 0.000000000000000000, 1.000000000000000000 ) ) ;
#114554=AXIS2_PLACEMENT_3D ( 'NONE', #21806, #61735, #99068 ) ;
#114555=AXIS2_PLACEMENT_3D ( 'NONE', #109360, #49183, #40655 ) ;
#114556=FACE_OUTER_BOUND ( 'NONE', #32271, .T. ) ;
#114557=EDGE_LOOP ( 'NONE', ( #55608, #6782, #106660, #128933 ) ) ;
#114558=AXIS2_PLACEMENT_3D ( 'NONE', #122639, #11384, #102985 ) ;
#114559=EDGE_LOOP ( 'NONE', ( #76055, #117809 ) ) ;
#114560=VERTEX_POINT ( 'NONE', #80828 ) ;
#114561=FACE_OUTER_BOUND ( 'NONE', #123770, .T. ) ;
#114562=AXIS2_PLACEMENT_3D ( 'NONE', #108698, #39346, #49800 ) ;
#114563=DIRECTION ( 'NONE',  ( 0.000000000000000000, 0.000000000000000000, -1.000000000000000000 ) ) ;
#114564=CARTESIAN_POINT ( 'NONE',  ( -9.200000000000009948, 12.50000000000000000, -4.330127018922197202 ) ) ;
#114565=ORIENTED_EDGE ( 'NONE', *, *, #26542, .T. ) ;
#114566=DIRECTION ( 'NONE',  ( 0.000000000000000000, 0.000000000000000000, -1.000000000000000000 ) ) ;
#114567=FACE_OUTER_BOUND ( 'NONE', #80371, .T. ) ;
#114568=CIRCLE ( 'NONE', #56084, 0.06509327318403745899 ) ;
#114569=DIRECTION ( 'NONE',  ( 0.000000000000000000, 1.000000000000000000, 0.000000000000000000 ) ) ;
#114570=FACE_OUTER_BOUND ( 'NONE', #96059, .T. ) ;
#114571=CARTESIAN_POINT ( 'NONE',  ( -6.650000000000015454, 12.50000000000000000, 2.857883832488649301 ) ) ;
#114572=EDGE_LOOP ( 'NONE', ( #69550, #83415, #63581, #32713 ) ) ;
#114573=CONICAL_SURFACE ( 'NONE', #89544, 0.1000000000000002554, 0.003490658503988666988 ) ;
#114574=AXIS2_PLACEMENT_3D ( 'NONE', #22368, #53105, #23633 ) ;
#114575=CARTESIAN_POINT ( 'NONE',  ( -10.85000000000000142, 2.500000000000000000, -5.902370205355746968 ) ) ;
#114576=ORIENTED_EDGE ( 'NONE', *, *, #75452, .F. ) ;
#114577=EDGE_LOOP ( 'NONE', ( #72697, #2091, #120577, #56 ) ) ;
#114578=ADVANCED_FACE ( 'NONE', ( #120738 ), #31094, .T. ) ;
#114579=CARTESIAN_POINT ( 'NONE',  ( -10.65000000000000213, 12.50000000000000000, 1.818653347947321475 ) ) ;
#114580=FACE_BOUND ( 'NONE', #59896, .T. ) ;
#114581=DIRECTION ( 'NONE',  ( 0.000000000000000000, 0.000000000000000000, -1.000000000000000000 ) ) ;
#114582=DIRECTION ( 'NONE',  ( 0.000000000000000000, 1.000000000000000000, 0.000000000000000000 ) ) ;
#114583=DIRECTION ( 'NONE',  ( 0.000000000000000000, 0.000000000000000000, -1.000000000000000000 ) ) ;
#114584=ORIENTED_EDGE ( 'NONE', *, *, #51055, .F. ) ;
#114585=EDGE_CURVE ( 'NONE', #26891, #76567, #21911, .T. ) ;
#114586=VECTOR ( 'NONE', #30926, 1000.000000000000000 ) ;
#114587=ORIENTED_EDGE ( 'NONE', *, *, #7831, .F. ) ;
#114588=ADVANCED_FACE ( 'NONE', ( #13990 ), #122039, .T. ) ;
#114589=DIRECTION ( 'NONE',  ( 0.000000000000000000, 0.000000000000000000, 1.000000000000000000 ) ) ;
#114590=DIRECTION ( 'NONE',  ( 0.000000000000000000, 0.000000000000000000, 1.000000000000000000 ) ) ;
#114591=CARTESIAN_POINT ( 'NONE',  ( 16.98389417445357452, -2.499999999999999556, -5.627887362461234666 ) ) ;
#114592=ADVANCED_FACE ( 'NONE', ( #113491 ), #72299, .T. ) ;
#114593=FACE_OUTER_BOUND ( 'NONE', #93058, .T. ) ;
#114594=ORIENTED_EDGE ( 'NONE', *, *, #91255, .T. ) ;
#114595=CARTESIAN_POINT ( 'NONE',  ( -12.29999999999999538, 12.50000000000000000, -4.676537180435976104 ) ) ;
#114596=CIRCLE ( 'NONE', #39425, 0.06509327318403745899 ) ;
#114597=DIRECTION ( 'NONE',  ( 0.000000000000000000, 0.000000000000000000, 1.000000000000000000 ) ) ;
#114598=AXIS2_PLACEMENT_3D ( 'NONE', #30, #30158, #81806 ) ;
#114599=EDGE_CURVE ( 'NONE', #100830, #42825, #44475, .T. ) ;
#114600=VERTEX_POINT ( 'NONE', #112214 ) ;
#114601=CARTESIAN_POINT ( 'NONE',  ( 10.44999999999991047, 2.500000000000000000, -6.495190528383302464 ) ) ;
#114602=EDGE_CURVE ( 'NONE', #79817, #93212, #22560, .T. ) ;
#114603=ORIENTED_EDGE ( 'NONE', *, *, #125950, .T. ) ;
#114604=FACE_BOUND ( 'NONE', #51409, .T. ) ;
#114605=FACE_OUTER_BOUND ( 'NONE', #17441, .T. ) ;
#114606=EDGE_CURVE ( 'NONE', #69532, #76244, #92569, .T. ) ;
#114607=AXIS2_PLACEMENT_3D ( 'NONE', #51750, #12448, #40004 ) ;
#114608=EDGE_CURVE ( 'NONE', #79956, #53157, #84176, .T. ) ;
#114610=VERTEX_POINT ( 'NONE', #23173 ) ;
#114611=DIRECTION ( 'NONE',  ( -0.000000000000000000, 1.000000000000000000, -0.000000000000000000 ) ) ;
#114612=DIRECTION ( 'NONE',  ( -0.000000000000000000, 1.000000000000000000, -0.000000000000000000 ) ) ;
#114613=ORIENTED_EDGE ( 'NONE', *, *, #20277, .F. ) ;
#114614=ORIENTED_EDGE ( 'NONE', *, *, #120078, .F. ) ;
#114616=EDGE_CURVE ( 'NONE', #55512, #20680, #4747, .T. ) ;
#114618=DIRECTION ( 'NONE',  ( -0.000000000000000000, 1.000000000000000000, -0.000000000000000000 ) ) ;
#114619=AXIS2_PLACEMENT_3D ( 'NONE', #72594, #61492, #22863 ) ;
#114620=CARTESIAN_POINT ( 'NONE',  ( 4.999999999999938716, 2.500000000000000000, -5.022947341949754119 ) ) ;
#114621=CARTESIAN_POINT ( 'NONE',  ( -6.700000000000016165, 12.50000000000000000, 4.330127018922196314 ) ) ;
#114622=FACE_OUTER_BOUND ( 'NONE', #87954, .T. ) ;
#114623=CARTESIAN_POINT ( 'NONE',  ( 0.6499999999999561684, 2.500000000000000000, 2.411473670974873862 ) ) ;
#114624=AXIS2_PLACEMENT_3D ( 'NONE', #64096, #82467, #14960 ) ;
#114626=ORIENTED_EDGE ( 'NONE', *, *, #10704, .F. ) ;
#114627=DIRECTION ( 'NONE',  ( -0.000000000000000000, 1.000000000000000000, -0.000000000000000000 ) ) ;
#114629=FACE_OUTER_BOUND ( 'NONE', #50115, .T. ) ;
#114630=AXIS2_PLACEMENT_3D ( 'NONE', #95083, #103621, #104879 ) ;
#114631=DIRECTION ( 'NONE',  ( -0.000000000000000000, -1.000000000000000000, -0.000000000000000000 ) ) ;
#114632=EDGE_LOOP ( 'NONE', ( #43649, #10544 ) ) ;
#114633=EDGE_LOOP ( 'NONE', ( #116119, #112356 ) ) ;
#114634=FACE_BOUND ( 'NONE', #115469, .T. ) ;
#114635=VERTEX_POINT ( 'NONE', #101749 ) ;
#114636=EDGE_CURVE ( 'NONE', #57530, #65577, #123951, .T. ) ;
#114637=FACE_OUTER_BOUND ( 'NONE', #105343, .T. ) ;
#114638=DIRECTION ( 'NONE',  ( -0.000000000000000000, 1.000000000000000000, -0.000000000000000000 ) ) ;
#114639=ORIENTED_EDGE ( 'NONE', *, *, #84591, .T. ) ;
#114640=FACE_OUTER_BOUND ( 'NONE', #82424, .T. ) ;
#114641=CIRCLE ( 'NONE', #47761, 0.06509327318403745899 ) ;
#114642=CARTESIAN_POINT ( 'NONE',  ( 5.649999999999936406, 2.500000000000000000, -6.048780366869526581 ) ) ;
#114643=CARTESIAN_POINT ( 'NONE',  ( -11.69999999999999929, 12.50000000000000000, -0.06509327318403569651 ) ) ;
#114644=DIRECTION ( 'NONE',  ( 0.000000000000000000, 0.000000000000000000, 1.000000000000000000 ) ) ;
#114646=CARTESIAN_POINT ( 'NONE',  ( 3.149999999999944400, 12.50000000000000000, 1.818653347947321475 ) ) ;
#114647=LINE ( 'NONE', #123816, #109071 ) ;
#114648=CARTESIAN_POINT ( 'NONE',  ( -10.20000000000000284, 2.500000000000000000, 3.983716857408420964 ) ) ;
#114649=PLANE ( 'NONE',  #38107 ) ;
#114650=CIRCLE ( 'NONE', #60308, 0.06509327318403745899 ) ;
#114651=DIRECTION ( 'NONE',  ( 0.000000000000000000, 0.000000000000000000, 1.000000000000000000 ) ) ;
#114652=ORIENTED_EDGE ( 'NONE', *, *, #116175, .T. ) ;
#114653=AXIS2_PLACEMENT_3D ( 'NONE', #91728, #80633, #60357 ) ;
#114654=ORIENTED_EDGE ( 'NONE', *, *, #98864, .F. ) ;
#114655=ADVANCED_FACE ( 'NONE', ( #34314 ), #48696, .T. ) ;
#114656=ORIENTED_EDGE ( 'NONE', *, *, #11073, .T. ) ;
#114657=FACE_OUTER_BOUND ( 'NONE', #22201, .T. ) ;
#114658=EDGE_LOOP ( 'NONE', ( #43627, #17942, #24866, #18493 ) ) ;
#114659=CARTESIAN_POINT ( 'NONE',  ( 9.549999999999915445, 2.500000000000000000, 6.395190528383296602 ) ) ;
#114660=EDGE_LOOP ( 'NONE', ( #950, #21169 ) ) ;
#114661=ORIENTED_EDGE ( 'NONE', *, *, #13826, .F. ) ;
#114662=EDGE_LOOP ( 'NONE', ( #30390, #81478, #21251, #24310 ) ) ;
#114663=AXIS2_PLACEMENT_3D ( 'NONE', #72162, #12568, #123808 ) ;
#114664=CARTESIAN_POINT ( 'NONE',  ( 10.64999999999991331, 12.50000000000000000, -2.511473670974877948 ) ) ;
#114665=DIRECTION ( 'NONE',  ( -0.000000000000000000, -1.000000000000000000, -0.000000000000000000 ) ) ;
#114666=DIRECTION ( 'NONE',  ( -0.000000000000000000, -1.000000000000000000, -0.000000000000000000 ) ) ;
#114667=DIRECTION ( 'NONE',  ( 0.000000000000000000, 0.000000000000000000, 1.000000000000000000 ) ) ;
#114668=DIRECTION ( 'NONE',  ( 0.000000000000000000, 0.000000000000000000, 1.000000000000000000 ) ) ;
#114669=CONICAL_SURFACE ( 'NONE', #81233, 0.1000000000000002554, 0.003490658503988666988 ) ;
#114670=ADVANCED_FACE ( 'NONE', ( #13352 ), #103690, .T. ) ;
#114671=VERTEX_POINT ( 'NONE', #53936 ) ;
#114672=CARTESIAN_POINT ( 'NONE',  ( -0.6500000000000389910, 12.50000000000000000, -1.818653347947326138 ) ) ;
#114673=ORIENTED_EDGE ( 'NONE', *, *, #16166, .F. ) ;
#114674=AXIS2_PLACEMENT_3D ( 'NONE', #6324, #77031, #16148 ) ;
#114675=VECTOR ( 'NONE', #94135, 1000.000000000000000 ) ;
#114676=ORIENTED_EDGE ( 'NONE', *, *, #46571, .F. ) ;
#114677=EDGE_LOOP ( 'NONE', ( #74552, #20061, #2007, #57157 ) ) ;
#114678=CARTESIAN_POINT ( 'NONE',  ( -4.150000000000024336, 12.50000000000000000, -2.099970236277064473 ) ) ;
#114679=ORIENTED_EDGE ( 'NONE', *, *, #29692, .F. ) ;
#114680=EDGE_LOOP ( 'NONE', ( #43240, #127652 ) ) ;
#114681=ORIENTED_EDGE ( 'NONE', *, *, #73935, .F. ) ;
#114682=DIRECTION ( 'NONE',  ( -0.000000000000000000, -1.000000000000000000, -0.000000000000000000 ) ) ;
#114683=CARTESIAN_POINT ( 'NONE',  ( -13.94999999999998863, 2.500000000000000000, -1.818653347947323917 ) ) ;
#114684=CARTESIAN_POINT ( 'NONE',  ( 8.149999999999920419, 12.50000000000000000, 6.841600689897072485 ) ) ;
#114685=CARTESIAN_POINT ( 'NONE',  ( -0.2000000000000399791, 12.50000000000000000, -4.676537180435977881 ) ) ;
#114686=PLANE ( 'NONE',  #118187 ) ;
#114687=CARTESIAN_POINT ( 'NONE',  ( -2.500000000000032863, 12.50000000000000000, 5.022947341949748790 ) ) ;
#114688=VERTEX_POINT ( 'NONE', #4166 ) ;
#114689=FACE_OUTER_BOUND ( 'NONE', #75228, .T. ) ;
#114690=VERTEX_POINT ( 'NONE', #52635 ) ;
#114691=AXIS2_PLACEMENT_3D ( 'NONE', #126973, #37313, #17644 ) ;
#114692=DIRECTION ( 'NONE',  ( 0.000000000000000000, 1.000000000000000000, 0.000000000000000000 ) ) ;
#114693=ADVANCED_FACE ( 'NONE', ( #2908 ), #126033, .T. ) ;
#114694=AXIS2_PLACEMENT_3D ( 'NONE', #13753, #94258, #86365 ) ;
#114695=ORIENTED_EDGE ( 'NONE', *, *, #91198, .F. ) ;
#114696=DIRECTION ( 'NONE',  ( -0.000000000000000000, 1.000000000000000000, -0.000000000000000000 ) ) ;
#114697=VECTOR ( 'NONE', #56072, 1000.000000000000000 ) ;
#114698=ORIENTED_EDGE ( 'NONE', *, *, #75702, .T. ) ;
#114699=ORIENTED_EDGE ( 'NONE', *, *, #107376, .T. ) ;
#114700=ADVANCED_FACE ( 'NONE', ( #82770 ), #46625, .T. ) ;
#114701=CONICAL_SURFACE ( 'NONE', #41578, 0.09999999999999982514, 0.003490658503988666988 ) ;
#114702=PLANE ( 'NONE',  #120100 ) ;
#114703=DIRECTION ( 'NONE',  ( 0.000000000000000000, 0.000000000000000000, 1.000000000000000000 ) ) ;
#114704=CIRCLE ( 'NONE', #95928, 0.06509327318403745899 ) ;
#114705=AXIS2_PLACEMENT_3D ( 'NONE', #45640, #64614, #46929 ) ;
#114706=DIRECTION ( 'NONE',  ( -0.000000000000000000, 1.000000000000000000, -0.000000000000000000 ) ) ;
#114707=ADVANCED_FACE ( 'NONE', ( #122670 ), #3543, .T. ) ;
#114708=CARTESIAN_POINT ( 'NONE',  ( -6.650000000000018119, 12.50000000000000000, -2.165063509461101710 ) ) ;
#114710=ORIENTED_EDGE ( 'NONE', *, *, #51603, .F. ) ;
#114711=DIRECTION ( 'NONE',  ( 0.000000000000000000, 0.000000000000000000, -1.000000000000000000 ) ) ;
#114712=CARTESIAN_POINT ( 'NONE',  ( -2.100000000000034728, 12.50000000000000000, 4.330127018922196314 ) ) ;
#114713=ADVANCED_FACE ( 'NONE', ( #116550 ), #121832, .T. ) ;
#114714=DIRECTION ( 'NONE',  ( 0.000000000000000000, 0.000000000000000000, 1.000000000000000000 ) ) ;
#114715=EDGE_CURVE ( 'NONE', #75618, #78396, #109310, .T. ) ;
#114716=EDGE_CURVE ( 'NONE', #116590, #126587, #90537, .T. ) ;
#114717=FACE_OUTER_BOUND ( 'NONE', #65730, .T. ) ;
#114718=LINE ( 'NONE', #7333, #121152 ) ;
#114719=CONICAL_SURFACE ( 'NONE', #12215, 0.1000000000000002554, 0.003490658503988666988 ) ;
#114720=VERTEX_POINT ( 'NONE', #37371 ) ;
#114721=EDGE_LOOP ( 'NONE', ( #44540, #33545 ) ) ;
#114722=ADVANCED_FACE ( 'NONE', ( #68092 ), #26892, .T. ) ;
#114724=ADVANCED_FACE ( 'NONE', ( #78591 ), #31978, .T. ) ;
#114725=DIRECTION ( 'NONE',  ( 0.000000000000000000, -0.000000000000000000, 1.000000000000000000 ) ) ;
#114726=CARTESIAN_POINT ( 'NONE',  ( -11.25000000000000000, 12.50000000000000000, 2.857883832488649301 ) ) ;
#114727=CONICAL_SURFACE ( 'NONE', #97996, 0.1000000000000002554, 0.003490658503988666988 ) ;
#114728=EDGE_CURVE ( 'NONE', #103358, #22461, #89036, .T. ) ;
#114729=CIRCLE ( 'NONE', #85491, 0.09999999999999999167 ) ;
#114731=CARTESIAN_POINT ( 'NONE',  ( 9.149999999999920419, 2.500000000000000000, -7.088010851410853519 ) ) ;
#114732=CARTESIAN_POINT ( 'NONE',  ( -7.700000000000014388, 12.50000000000000000, -4.741630453620015118 ) ) ;
#114733=LINE ( 'NONE', #83359, #48146 ) ;
#114734=LINE ( 'NONE', #45372, #118630 ) ;
#114735=EDGE_LOOP ( 'NONE', ( #53706, #27959 ) ) ;
#114736=CARTESIAN_POINT ( 'NONE',  ( 7.699999999999923794, 2.500000000000000000, -0.3464101615137783474 ) ) ;
#114737=DIRECTION ( 'NONE',  ( 0.000000000000000000, 1.000000000000000000, 0.000000000000000000 ) ) ;
#114738=CONICAL_SURFACE ( 'NONE', #129443, 0.1000000000000002554, 0.003490658503988666988 ) ;
#114739=ORIENTED_EDGE ( 'NONE', *, *, #69967, .F. ) ;
#114740=AXIS2_PLACEMENT_3D ( 'NONE', #96475, #116129, #66388 ) ;
#114741=DIRECTION ( 'NONE',  ( 0.000000000000000000, 0.000000000000000000, -1.000000000000000000 ) ) ;
#114742=CIRCLE ( 'NONE', #89623, 0.06509327318403745899 ) ;
#114743=ORIENTED_EDGE ( 'NONE', *, *, #79398, .T. ) ;
#114744=DIRECTION ( 'NONE',  ( 0.000000000000000000, 0.000000000000000000, 1.000000000000000000 ) ) ;
#114745=ORIENTED_EDGE ( 'NONE', *, *, #76474, .F. ) ;
#114746=DIRECTION ( 'NONE',  ( 0.000000000000000000, 0.000000000000000000, 1.000000000000000000 ) ) ;
#114747=CIRCLE ( 'NONE', #54122, 9.000000000000001776 ) ;
#114748=CARTESIAN_POINT ( 'NONE',  ( 0.4499999999999569344, 2.500000000000000000, 2.165063509461097713 ) ) ;
#114749=LINE ( 'NONE', #15242, #6703 ) ;
#114750=ORIENTED_EDGE ( 'NONE', *, *, #69459, .T. ) ;
#114751=CARTESIAN_POINT ( 'NONE',  ( -11.05000000000000249, 2.500000000000000000, -1.818653347947322141 ) ) ;
#114752=CIRCLE ( 'NONE', #58351, 0.06509327318403741736 ) ;
#114753=CONICAL_SURFACE ( 'NONE', #123089, 0.1000000000000000472, 0.003490658503988666988 ) ;
#114755=AXIS2_PLACEMENT_3D ( 'NONE', #26584, #35756, #46873 ) ;
#114756=ADVANCED_FACE ( 'NONE', ( #87728 ), #111465, .T. ) ;
#114757=VERTEX_POINT ( 'NONE', #66795 ) ;
#114758=FACE_OUTER_BOUND ( 'NONE', #83495, .T. ) ;
#114759=ADVANCED_FACE ( 'NONE', ( #128986 ), #61305, .T. ) ;
#114760=CIRCLE ( 'NONE', #43786, 0.09999999999999982514 ) ;
#114761=AXIS2_PLACEMENT_3D ( 'NONE', #111020, #100570, #60038 ) ;
#114762=ORIENTED_EDGE ( 'NONE', *, *, #114298, .F. ) ;
#114763=EDGE_CURVE ( 'NONE', #48350, #70125, #58933, .T. ) ;
#114764=VERTEX_POINT ( 'NONE', #119137 ) ;
#114765=PLANE ( 'NONE',  #65166 ) ;
#114766=CARTESIAN_POINT ( 'NONE',  ( 8.549999999999920774, 2.500000000000000000, -2.511473670974877948 ) ) ;
#114767=EDGE_LOOP ( 'NONE', ( #62476, #81613, #54802, #31399 ) ) ;
#114768=CARTESIAN_POINT ( 'NONE',  ( 3.349999999999945466, 12.50000000000000000, -2.230156782645139391 ) ) ;
#114769=DIRECTION ( 'NONE',  ( 0.000000000000000000, 0.000000000000000000, -1.000000000000000000 ) ) ;
#114770=VERTEX_POINT ( 'NONE', #98840 ) ;
#114771=EDGE_CURVE ( 'NONE', #59538, #12415, #9182, .T. ) ;
#114772=DIRECTION ( 'NONE',  ( 0.000000000000000000, 1.000000000000000000, 0.000000000000000000 ) ) ;
#114773=DIRECTION ( 'NONE',  ( 0.000000000000000000, 0.000000000000000000, 1.000000000000000000 ) ) ;
#114774=DIRECTION ( 'NONE',  ( -0.000000000000000000, -1.000000000000000000, -0.000000000000000000 ) ) ;
#114775=CONICAL_SURFACE ( 'NONE', #49973, 0.1000000000000002554, 0.003490658503988666988 ) ;
#114776=DIRECTION ( 'NONE',  ( -0.000000000000000000, 1.000000000000000000, -0.000000000000000000 ) ) ;
#114777=DIRECTION ( 'NONE',  ( -4.274815082592931898E-19, -0.9999939076577903929, -0.003490651415223739937 ) ) ;
#114778=CARTESIAN_POINT ( 'NONE',  ( 15.39999999999989200, 2.500000000000000000, 0.6928203230275494784 ) ) ;
#114779=CIRCLE ( 'NONE', #33344, 0.1000000000000000472 ) ;
#114780=AXIS2_PLACEMENT_3D ( 'NONE', #44513, #84448, #124377 ) ;
#114781=ORIENTED_EDGE ( 'NONE', *, *, #10468, .T. ) ;
#114782=VERTEX_POINT ( 'NONE', #19653 ) ;
#114783=EDGE_LOOP ( 'NONE', ( #20885, #63961 ) ) ;
#114784=ORIENTED_EDGE ( 'NONE', *, *, #62445, .F. ) ;
#114785=CARTESIAN_POINT ( 'NONE',  ( -10.65000000000000391, 2.500000000000000000, -6.248780366869523206 ) ) ;
#114786=CARTESIAN_POINT ( 'NONE',  ( 2.899999999999946620, 2.500000000000000000, -0.7928203230275543412 ) ) ;
#114787=LINE ( 'NONE', #85336, #2972 ) ;
#114788=VERTEX_POINT ( 'NONE', #79225 ) ;
#114789=FACE_BOUND ( 'NONE', #81107, .T. ) ;
#114790=ADVANCED_FACE ( 'NONE', ( #29471 ), #21587, .T. ) ;
#114791=FACE_OUTER_BOUND ( 'NONE', #43788, .T. ) ;
#114792=CARTESIAN_POINT ( 'NONE',  ( -1.850000000000033396, 2.500000000000000000, -6.741600689897077281 ) ) ;
#114793=CIRCLE ( 'NONE', #70896, 0.06509327318403745899 ) ;
#114794=AXIS2_PLACEMENT_3D ( 'NONE', #96640, #16786, #75724 ) ;
#114795=CARTESIAN_POINT ( 'NONE',  ( -0.4500000000000397571, 12.50000000000000000, -2.230156782645139391 ) ) ;
#114796=AXIS2_PLACEMENT_3D ( 'NONE', #43220, #33399, #81823 ) ;
#114797=DIRECTION ( 'NONE',  ( 0.000000000000000000, -0.000000000000000000, 1.000000000000000000 ) ) ;
#114798=CARTESIAN_POINT ( 'NONE',  ( 10.59999999999990905, 2.500000000000000000, 4.676537180435972552 ) ) ;
#114799=CARTESIAN_POINT ( 'NONE',  ( -2.700000000000030376, 2.500000000000000000, 3.983716857408420964 ) ) ;
#114800=FACE_OUTER_BOUND ( 'NONE', #56733, .T. ) ;
#114801=DIRECTION ( 'NONE',  ( 0.000000000000000000, -0.000000000000000000, 1.000000000000000000 ) ) ;
#114802=CARTESIAN_POINT ( 'NONE',  ( -0.2000000000000347888, 2.500000000000000000, 0.4464101615137758272 ) ) ;
#114803=AXIS2_PLACEMENT_3D ( 'NONE', #85939, #18502, #77426 ) ;
#114804=DIRECTION ( 'NONE',  ( -0.000000000000000000, 1.000000000000000000, -0.000000000000000000 ) ) ;
#114805=AXIS2_PLACEMENT_3D ( 'NONE', #75124, #115032, #54826 ) ;
#114806=ORIENTED_EDGE ( 'NONE', *, *, #22038, .T. ) ;
#114807=ORIENTED_EDGE ( 'NONE', *, *, #52627, .F. ) ;
#114808=EDGE_CURVE ( 'NONE', #22187, #76885, #30423, .T. ) ;
#114809=EDGE_LOOP ( 'NONE', ( #76895, #121204 ) ) ;
#114810=VERTEX_POINT ( 'NONE', #42531 ) ;
#114811=DIRECTION ( 'NONE',  ( 0.000000000000000000, 0.000000000000000000, 1.000000000000000000 ) ) ;
#114812=ORIENTED_EDGE ( 'NONE', *, *, #13342, .T. ) ;
#114813=ORIENTED_EDGE ( 'NONE', *, *, #32775, .F. ) ;
#114814=VERTEX_POINT ( 'NONE', #82454 ) ;
#114815=FACE_OUTER_BOUND ( 'NONE', #77697, .T. ) ;
#114816=DIRECTION ( 'NONE',  ( 0.000000000000000000, 1.000000000000000000, 0.000000000000000000 ) ) ;
#114817=CARTESIAN_POINT ( 'NONE',  ( 12.89999999999990266, 2.500000000000000000, -3.637306695894650055 ) ) ;
#114818=CIRCLE ( 'NONE', #104366, 0.1000000000000002554 ) ;
#114819=DIRECTION ( 'NONE',  ( -0.000000000000000000, -1.000000000000000000, -0.000000000000000000 ) ) ;
#114820=EDGE_CURVE ( 'NONE', #87351, #64508, #63360, .T. ) ;
#114821=EDGE_LOOP ( 'NONE', ( #18087, #123051, #10028, #18211 ) ) ;
#114822=ORIENTED_EDGE ( 'NONE', *, *, #33166, .T. ) ;
#114823=ORIENTED_EDGE ( 'NONE', *, *, #4604, .T. ) ;
#114824=DIRECTION ( 'NONE',  ( 0.000000000000000000, 0.000000000000000000, 1.000000000000000000 ) ) ;
#114825=EDGE_LOOP ( 'NONE', ( #112147, #1222 ) ) ;
#114826=DIRECTION ( 'NONE',  ( 0.000000000000000000, 1.000000000000000000, 0.000000000000000000 ) ) ;
#114827=ORIENTED_EDGE ( 'NONE', *, *, #94095, .T. ) ;
#114829=AXIS2_PLACEMENT_3D ( 'NONE', #29694, #68968, #108878 ) ;
#114830=CARTESIAN_POINT ( 'NONE',  ( 1.649999999999951505, 2.500000000000000000, 1.472243186433545459 ) ) ;
#114831=DIRECTION ( 'NONE',  ( -0.000000000000000000, 1.000000000000000000, -0.000000000000000000 ) ) ;
#114832=DIRECTION ( 'NONE',  ( -4.274815082592931898E-19, -0.9999939076577903929, -0.003490651415223739937 ) ) ;
#114833=CARTESIAN_POINT ( 'NONE',  ( -5.600000000000020073, 2.500000000000000000, -0.3464101615137782364 ) ) ;
#114834=CARTESIAN_POINT ( 'NONE',  ( 6.699999999999928235, 12.50000000000000000, -2.276824562219559311E-15 ) ) ;
#114835=CIRCLE ( 'NONE', #62635, 0.1000000000000002554 ) ;
#114836=ORIENTED_EDGE ( 'NONE', *, *, #123821, .T. ) ;
#114838=ORIENTED_EDGE ( 'NONE', *, *, #16646, .T. ) ;
#114839=DIRECTION ( 'NONE',  ( 0.000000000000000000, 1.000000000000000000, 0.000000000000000000 ) ) ;
#114840=EDGE_CURVE ( 'NONE', #890, #59538, #71766, .T. ) ;
#114841=AXIS2_PLACEMENT_3D ( 'NONE', #107805, #27296, #117593 ) ;
#114842=AXIS2_PLACEMENT_3D ( 'NONE', #22064, #61982, #110423 ) ;
#114843=EDGE_LOOP ( 'NONE', ( #94962, #3577 ) ) ;
#114844=LINE ( 'NONE', #13424, #29603 ) ;
#114845=DIRECTION ( 'NONE',  ( 0.000000000000000000, -0.9999939076577903929, 0.003490651415223739937 ) ) ;
#114846=AXIS2_PLACEMENT_3D ( 'NONE', #11286, #128525, #80035 ) ;
#114847=DIRECTION ( 'NONE',  ( 0.000000000000000000, 0.000000000000000000, 1.000000000000000000 ) ) ;
#114848=DIRECTION ( 'NONE',  ( 0.000000000000000000, -0.000000000000000000, 1.000000000000000000 ) ) ;
#114849=ORIENTED_EDGE ( 'NONE', *, *, #31583, .F. ) ;
#114850=EDGE_CURVE ( 'NONE', #77606, #90795, #88475, .T. ) ;
#114852=VECTOR ( 'NONE', #78990, 1000.000000000000000 ) ;
#114853=CIRCLE ( 'NONE', #45925, 0.1000000000000000472 ) ;
#114854=DIRECTION ( 'NONE',  ( 0.000000000000000000, 0.000000000000000000, -1.000000000000000000 ) ) ;
#114855=EDGE_LOOP ( 'NONE', ( #56605, #46027 ) ) ;
#114856=ORIENTED_EDGE ( 'NONE', *, *, #82991, .F. ) ;
#114857=EDGE_CURVE ( 'NONE', #110459, #75028, #34116, .T. ) ;
#114858=ADVANCED_FACE ( 'NONE', ( #12395 ), #84278, .T. ) ;
#114859=EDGE_LOOP ( 'NONE', ( #114990, #65128, #84259, #113399 ) ) ;
#114860=CARTESIAN_POINT ( 'NONE',  ( 12.09999999999990550, 2.500000000000000000, -5.022947341949754119 ) ) ;
#114861=PLANE ( 'NONE',  #70089 ) ;
#114862=EDGE_CURVE ( 'NONE', #30008, #115201, #70679, .T. ) ;
#114864=EDGE_CURVE ( 'NONE', #59594, #3679, #27840, .T. ) ;
#114865=DIRECTION ( 'NONE',  ( 0.000000000000000000, 0.000000000000000000, 1.000000000000000000 ) ) ;
#114866=DIRECTION ( 'NONE',  ( -0.000000000000000000, -1.000000000000000000, -0.000000000000000000 ) ) ;
#114867=DIRECTION ( 'NONE',  ( -0.000000000000000000, -1.000000000000000000, -0.000000000000000000 ) ) ;
#114869=CIRCLE ( 'NONE', #89748, 0.09999999999999982514 ) ;
#114870=EDGE_CURVE ( 'NONE', #87504, #18257, #1290, .T. ) ;
#114871=EDGE_CURVE ( 'NONE', #50596, #103587, #71312, .T. ) ;
#114872=ORIENTED_EDGE ( 'NONE', *, *, #60526, .F. ) ;
#114873=ADVANCED_FACE ( 'NONE', ( #102079 ), #44574, .T. ) ;
#114874=DIRECTION ( 'NONE',  ( -0.000000000000000000, -1.000000000000000000, -0.000000000000000000 ) ) ;
#114875=EDGE_CURVE ( 'NONE', #6351, #77555, #92240, .T. ) ;
#114876=AXIS2_PLACEMENT_3D ( 'NONE', #18115, #97968, #37771 ) ;
#114877=ORIENTED_EDGE ( 'NONE', *, *, #87349, .F. ) ;
#114878=DIRECTION ( 'NONE',  ( -0.000000000000000000, -1.000000000000000000, -0.000000000000000000 ) ) ;
#114879=CARTESIAN_POINT ( 'NONE',  ( -6.050000000000020250, 2.500000000000000000, -2.611473670974877592 ) ) ;
#114880=CARTESIAN_POINT ( 'NONE',  ( -0.8500000000000382805, 2.500000000000000000, -2.857883832488653741 ) ) ;
#114881=EDGE_CURVE ( 'NONE', #97225, #9827, #96785, .T. ) ;
#114882=VERTEX_POINT ( 'NONE', #111224 ) ;
#114883=VECTOR ( 'NONE', #90053, 1000.000000000000000 ) ;
#114884=AXIS2_PLACEMENT_3D ( 'NONE', #78642, #79908, #70097 ) ;
#114885=VECTOR ( 'NONE', #35959, 1000.000000000000000 ) ;
#114886=DIRECTION ( 'NONE',  ( -0.000000000000000000, -1.000000000000000000, -0.000000000000000000 ) ) ;
#114887=DIRECTION ( 'NONE',  ( -4.274815082592931898E-19, -0.9999939076577903929, -0.003490651415223739937 ) ) ;
#114888=CIRCLE ( 'NONE', #31302, 0.1000000000000002554 ) ;
#114889=EDGE_LOOP ( 'NONE', ( #27502, #115228 ) ) ;
#114890=CARTESIAN_POINT ( 'NONE',  ( 4.799999999999937650, 12.50000000000000000, -0.3464101615137782364 ) ) ;
#114891=AXIS2_PLACEMENT_3D ( 'NONE', #109589, #8780, #118748 ) ;
#114892=CIRCLE ( 'NONE', #75199, 0.06509327318403745899 ) ;
#114893=ORIENTED_EDGE ( 'NONE', *, *, #70418, .F. ) ;
#114894=VERTEX_POINT ( 'NONE', #70043 ) ;
#114895=DIRECTION ( 'NONE',  ( 0.000000000000000000, 1.000000000000000000, 0.000000000000000000 ) ) ;
#114896=VERTEX_POINT ( 'NONE', #62166 ) ;
#114897=PLANE ( 'NONE',  #107095 ) ;
#114898=CARTESIAN_POINT ( 'NONE',  ( -12.69999999999999396, 2.500000000000000000, 0.2464101615137776757 ) ) ;
#114899=AXIS2_PLACEMENT_3D ( 'NONE', #85763, #66130, #6527 ) ;
#114900=CARTESIAN_POINT ( 'NONE',  ( -4.999999999999990230, 12.50000000000000000, -4.330127018922201643 ) ) ;
#114901=ORIENTED_EDGE ( 'NONE', *, *, #93885, .T. ) ;
#114902=FACE_BOUND ( 'NONE', #126735, .T. ) ;
#114903=DIRECTION ( 'NONE',  ( 0.000000000000000000, 0.000000000000000000, -1.000000000000000000 ) ) ;
#114904=VERTEX_POINT ( 'NONE', #121704 ) ;
#114905=CARTESIAN_POINT ( 'NONE',  ( -8.150000000000009237, 2.500000000000000000, 6.048780366869520364 ) ) ;
#114906=DIRECTION ( 'NONE',  ( -0.000000000000000000, 1.000000000000000000, -0.000000000000000000 ) ) ;
#114907=ORIENTED_EDGE ( 'NONE', *, *, #70691, .F. ) ;
#114908=ADVANCED_FACE ( 'NONE', ( #2557 ), #32072, .T. ) ;
#114909=ORIENTED_EDGE ( 'NONE', *, *, #29479, .T. ) ;
#114910=EDGE_CURVE ( 'NONE', #1125, #103358, #80085, .T. ) ;
#114911=ORIENTED_EDGE ( 'NONE', *, *, #45150, .F. ) ;
#114912=CARTESIAN_POINT ( 'NONE',  ( -10.85000000000000142, 2.500000000000000000, -1.372243186433546036 ) ) ;
#114913=CARTESIAN_POINT ( 'NONE',  ( 2.500000000000002220, 2.499999999999999556, 10.00000000000000533 ) ) ;
#114914=ADVANCED_FACE ( 'NONE', ( #89678 ), #31753, .T. ) ;
#114915=LINE ( 'NONE', #14762, #31662 ) ;
#114916=FACE_BOUND ( 'NONE', #1934, .T. ) ;
#114917=ORIENTED_EDGE ( 'NONE', *, *, #32708, .F. ) ;
#114919=CARTESIAN_POINT ( 'NONE',  ( 10.79999999999991367, 12.50000000000000000, -0.06509327318403980434 ) ) ;
#114920=CARTESIAN_POINT ( 'NONE',  ( 7.099999999999927702, 2.500000000000000000, -3.737306695894649700 ) ) ;
#114921=ADVANCED_FACE ( 'NONE', ( #90298 ), #80391, .T. ) ;
#114922=DIRECTION ( 'NONE',  ( -0.000000000000000000, -1.000000000000000000, -0.000000000000000000 ) ) ;
#114923=ADVANCED_FACE ( 'NONE', ( #85000 ), #115665, .T. ) ;
#114924=CARTESIAN_POINT ( 'NONE',  ( -2.499999999999996003, 2.500000000000000000, -4.230127018922201998 ) ) ;
#114925=CARTESIAN_POINT ( 'NONE',  ( -10.60000000000000142, 2.500000000000000000, -0.2464101615137782308 ) ) ;
#114926=CONICAL_SURFACE ( 'NONE', #6251, 0.1000000000000000472, 0.003490658503988666988 ) ;
#114927=DIRECTION ( 'NONE',  ( 0.000000000000000000, 1.000000000000000000, 0.000000000000000000 ) ) ;
#114928=CARTESIAN_POINT ( 'NONE',  ( -4.600000000000028955, 12.50000000000000000, -4.265033745738164406 ) ) ;
#114930=CIRCLE ( 'NONE', #62736, 0.06509327318403745899 ) ;
#114931=CONICAL_SURFACE ( 'NONE', #75236, 0.1000000000000002554, 0.003490658503988666988 ) ;
#114933=VERTEX_POINT ( 'NONE', #5781 ) ;
#114934=ORIENTED_EDGE ( 'NONE', *, *, #56333, .T. ) ;
#114935=EDGE_LOOP ( 'NONE', ( #122074, #69014 ) ) ;
#114936=ORIENTED_EDGE ( 'NONE', *, *, #67268, .F. ) ;
#114938=CARTESIAN_POINT ( 'NONE',  ( -0.4000000000000331624, 2.500000000000000000, 0.1000000000000000056 ) ) ;
#114939=ORIENTED_EDGE ( 'NONE', *, *, #25022, .T. ) ;
#114940=FACE_BOUND ( 'NONE', #128797, .T. ) ;
#114941=LINE ( 'NONE', #13521, #89640 ) ;
#114942=AXIS2_PLACEMENT_3D ( 'NONE', #88336, #98173, #28156 ) ;
#114943=DIRECTION ( 'NONE',  ( 0.000000000000000000, 1.000000000000000000, 0.000000000000000000 ) ) ;
#114944=ORIENTED_EDGE ( 'NONE', *, *, #877, .F. ) ;
#114945=CARTESIAN_POINT ( 'NONE',  ( -7.050000000000013145, 2.500000000000000000, 6.595190528383296780 ) ) ;
#114946=DIRECTION ( 'NONE',  ( 0.000000000000000000, -0.9999939076577903929, 0.003490651415223739937 ) ) ;
#114947=DIRECTION ( 'NONE',  ( -0.000000000000000000, 1.000000000000000000, -0.000000000000000000 ) ) ;
#114948=ORIENTED_EDGE ( 'NONE', *, *, #103180, .F. ) ;
#114949=CARTESIAN_POINT ( 'NONE',  ( 3.749999999999938716, 2.500000000000000000, 7.188010851410848723 ) ) ;
#114950=EDGE_CURVE ( 'NONE', #69772, #118395, #9061, .T. ) ;
#114951=ORIENTED_EDGE ( 'NONE', *, *, #26743, .T. ) ;
#114952=EDGE_LOOP ( 'NONE', ( #92379, #33758, #15973, #56970 ) ) ;
#114953=EDGE_LOOP ( 'NONE', ( #90641, #101779 ) ) ;
#114954=CARTESIAN_POINT ( 'NONE',  ( 10.84999999999991260, 2.500000000000000000, -1.372243186433550033 ) ) ;
#114955=LINE ( 'NONE', #33830, #14252 ) ;
#114956=DIRECTION ( 'NONE',  ( 0.000000000000000000, 1.000000000000000000, 0.000000000000000000 ) ) ;
#114957=ORIENTED_EDGE ( 'NONE', *, *, #70740, .T. ) ;
#114958=CARTESIAN_POINT ( 'NONE',  ( 10.28037028461878855, 1.500000000000063283, -9.136909653556553934 ) ) ;
#114959=CIRCLE ( 'NONE', #18825, 0.06509327318403745899 ) ;
#114960=CARTESIAN_POINT ( 'NONE',  ( -0.6000000000000388356, 2.500000000000000000, 4.576537180435972019 ) ) ;
#114961=CONICAL_SURFACE ( 'NONE', #58559, 0.1000000000000002554, 0.003490658503988666988 ) ;
#114962=DIRECTION ( 'NONE',  ( -4.274815082592931898E-19, -0.9999939076577903929, -0.003490651415223739937 ) ) ;
#114964=CARTESIAN_POINT ( 'NONE',  ( 6.249999999999934275, 2.500000000000000000, -7.088010851410853519 ) ) ;
#114965=EDGE_CURVE ( 'NONE', #59645, #121477, #23750, .T. ) ;
#114966=CARTESIAN_POINT ( 'NONE',  ( 3.949999999999939782, 2.500000000000000000, 2.511473670974873507 ) ) ;
#114967=EDGE_CURVE ( 'NONE', #55845, #123356, #52975, .T. ) ;
#114968=VERTEX_POINT ( 'NONE', #85652 ) ;
#114969=CARTESIAN_POINT ( 'NONE',  ( -6.850000000000013856, 2.500000000000000000, 6.148780366869520897 ) ) ;
#114970=CIRCLE ( 'NONE', #87783, 0.06509327318403745899 ) ;
#114971=ORIENTED_EDGE ( 'NONE', *, *, #2226, .T. ) ;
#114972=ORIENTED_EDGE ( 'NONE', *, *, #41562, .F. ) ;
#114973=DIRECTION ( 'NONE',  ( 0.000000000000000000, 1.000000000000000000, 0.000000000000000000 ) ) ;
#114974=DIRECTION ( 'NONE',  ( 0.000000000000000000, 0.000000000000000000, 1.000000000000000000 ) ) ;
#114975=DIRECTION ( 'NONE',  ( 0.000000000000000000, 0.000000000000000000, -1.000000000000000000 ) ) ;
#114976=DIRECTION ( 'NONE',  ( -0.000000000000000000, 1.000000000000000000, -0.000000000000000000 ) ) ;
#114977=ADVANCED_FACE ( 'NONE', ( #24160 ), #61406, .T. ) ;
#114978=DIRECTION ( 'NONE',  ( 0.000000000000000000, 1.000000000000000000, 0.000000000000000000 ) ) ;
#114979=AXIS2_PLACEMENT_3D ( 'NONE', #112384, #113015, #33193 ) ;
#114980=EDGE_LOOP ( 'NONE', ( #92543, #104202, #86294, #114408 ) ) ;
#114981=ORIENTED_EDGE ( 'NONE', *, *, #70127, .F. ) ;
#114982=AXIS2_PLACEMENT_3D ( 'NONE', #63709, #12014, #62427 ) ;
#114983=DIRECTION ( 'NONE',  ( 0.000000000000000000, 0.000000000000000000, 1.000000000000000000 ) ) ;
#114984=DIRECTION ( 'NONE',  ( 0.000000000000000000, 0.000000000000000000, -1.000000000000000000 ) ) ;
#114985=CARTESIAN_POINT ( 'NONE',  ( -0.4000000000000392131, 2.500000000000000000, -4.230127018922201998 ) ) ;
#114986=ORIENTED_EDGE ( 'NONE', *, *, #99826, .T. ) ;
#114987=VERTEX_POINT ( 'NONE', #113834 ) ;
#114988=LINE ( 'NONE', #6312, #106297 ) ;
#114989=VECTOR ( 'NONE', #121675, 1000.000000000000000 ) ;
#114990=ORIENTED_EDGE ( 'NONE', *, *, #41614, .F. ) ;
#114991=CARTESIAN_POINT ( 'NONE',  ( -6.450000000000016165, 2.500000000000000000, 6.841600689897072485 ) ) ;
#114992=DIRECTION ( 'NONE',  ( -0.000000000000000000, -1.000000000000000000, -0.000000000000000000 ) ) ;
#114994=FACE_OUTER_BOUND ( 'NONE', #127990, .T. ) ;
#114995=CARTESIAN_POINT ( 'NONE',  ( 3.949999999999942446, 2.500000000000000000, -2.511473670974877948 ) ) ;
#114996=AXIS2_PLACEMENT_3D ( 'NONE', #86433, #117817, #57635 ) ;
#114997=CARTESIAN_POINT ( 'NONE',  ( -12.49999999999999467, 2.500000000000000000, -3.637306695894647390 ) ) ;
#114998=CARTESIAN_POINT ( 'NONE',  ( -8.950000000000008171, 2.500000000000000000, -2.511473670974877948 ) ) ;
#114999=ORIENTED_EDGE ( 'NONE', *, *, #1594, .T. ) ;
#115000=EDGE_CURVE ( 'NONE', #3252, #47024, #64082, .T. ) ;
#115001=CARTESIAN_POINT ( 'NONE',  ( 12.89999999999989733, 12.50000000000000000, 0.06509327318403504425 ) ) ;
#115002=CARTESIAN_POINT ( 'NONE',  ( 1.849999999999950129, 12.50000000000000000, -6.906693963081115939 ) ) ;
#115003=ORIENTED_EDGE ( 'NONE', *, *, #98575, .F. ) ;
#115004=EDGE_LOOP ( 'NONE', ( #98176, #102447 ) ) ;
#115005=EDGE_CURVE ( 'NONE', #2985, #53227, #73906, .T. ) ;
#115006=CARTESIAN_POINT ( 'NONE',  ( 6.449999999999931788, 2.500000000000000000, -2.511473670974877948 ) ) ;
#115007=CARTESIAN_POINT ( 'NONE',  ( 10.59999999999990905, 2.500000000000000000, 3.983716857408420076 ) ) ;
#115008=ADVANCED_FACE ( 'NONE', ( #34647 ), #86416, .T. ) ;
#115009=DIRECTION ( 'NONE',  ( -0.000000000000000000, -1.000000000000000000, -0.000000000000000000 ) ) ;
#115010=ADVANCED_FACE ( 'NONE', ( #76490 ), #111561, .T. ) ;
#115011=DIRECTION ( 'NONE',  ( 0.000000000000000000, -0.000000000000000000, 1.000000000000000000 ) ) ;
#115012=CARTESIAN_POINT ( 'NONE',  ( 11.64999999999990621, 2.500000000000000000, 6.495190528383297135 ) ) ;
#115013=LINE ( 'NONE', #93464, #90629 ) ;
#115014=DIRECTION ( 'NONE',  ( 0.000000000000000000, -0.9999939076577903929, 0.003490651415223739937 ) ) ;
#115015=DIRECTION ( 'NONE',  ( -0.000000000000000000, -1.000000000000000000, -0.000000000000000000 ) ) ;
#115016=DIRECTION ( 'NONE',  ( 0.000000000000000000, 0.000000000000000000, 1.000000000000000000 ) ) ;
#115017=EDGE_CURVE ( 'NONE', #89806, #82531, #105305, .T. ) ;
#115018=VECTOR ( 'NONE', #45637, 1000.000000000000000 ) ;
#115019=EDGE_CURVE ( 'NONE', #120570, #89280, #16871, .T. ) ;
#115020=AXIS2_PLACEMENT_3D ( 'NONE', #45634, #85539, #125463 ) ;
#115021=EDGE_CURVE ( 'NONE', #3965, #76244, #57185, .T. ) ;
#115022=DIRECTION ( 'NONE',  ( 0.000000000000000000, 0.000000000000000000, -1.000000000000000000 ) ) ;
#115023=VERTEX_POINT ( 'NONE', #96112 ) ;
#115024=CONICAL_SURFACE ( 'NONE', #125499, 0.1000000000000002554, 0.003490658503988666988 ) ;
#115025=AXIS2_PLACEMENT_3D ( 'NONE', #42180, #12690, #82096 ) ;
#115026=EDGE_CURVE ( 'NONE', #88347, #115125, #107868, .T. ) ;
#115027=VERTEX_POINT ( 'NONE', #57490 ) ;
#115028=EDGE_LOOP ( 'NONE', ( #65537, #79290 ) ) ;
#115029=ADVANCED_FACE ( 'NONE', ( #128166 ), #87576, .T. ) ;
#115031=DIRECTION ( 'NONE',  ( 0.000000000000000000, 0.000000000000000000, 1.000000000000000000 ) ) ;
#115032=DIRECTION ( 'NONE',  ( -0.000000000000000000, 1.000000000000000000, -0.000000000000000000 ) ) ;
#115033=ADVANCED_FACE ( 'NONE', ( #127517 ), #96883, .T. ) ;
#115034=ORIENTED_EDGE ( 'NONE', *, *, #62798, .F. ) ;
#115035=DIRECTION ( 'NONE',  ( 0.000000000000000000, 1.000000000000000000, 0.000000000000000000 ) ) ;
#115036=CARTESIAN_POINT ( 'NONE',  ( -6.050000000000018474, 2.500000000000000000, 6.841600689897072485 ) ) ;
#115037=PLANE ( 'NONE',  #14632 ) ;
#115038=ORIENTED_EDGE ( 'NONE', *, *, #90945, .F. ) ;
#115039=DIRECTION ( 'NONE',  ( -0.000000000000000000, 1.000000000000000000, -0.000000000000000000 ) ) ;
#115040=ORIENTED_EDGE ( 'NONE', *, *, #71569, .F. ) ;
#115041=EDGE_LOOP ( 'NONE', ( #71079, #36887, #88203, #47472 ) ) ;
#115042=EDGE_LOOP ( 'NONE', ( #102555, #117138 ) ) ;
#115043=VERTEX_POINT ( 'NONE', #98048 ) ;
#115044=CARTESIAN_POINT ( 'NONE',  ( -8.100000000000013856, 2.500000000000000000, -4.776537180435977525 ) ) ;
#115045=CARTESIAN_POINT ( 'NONE',  ( 9.599999999999917932, 12.50000000000000000, 0.06509327318403515528 ) ) ;
#115046=DIRECTION ( 'NONE',  ( 0.000000000000000000, -0.000000000000000000, 1.000000000000000000 ) ) ;
#115047=DIRECTION ( 'NONE',  ( 0.000000000000000000, 0.000000000000000000, 1.000000000000000000 ) ) ;
#115048=CIRCLE ( 'NONE', #64972, 0.1000000000000002554 ) ;
#115049=EDGE_LOOP ( 'NONE', ( #30869, #99677, #86748, #12670 ) ) ;
#115050=FACE_OUTER_BOUND ( 'NONE', #95035, .T. ) ;
#115051=ORIENTED_EDGE ( 'NONE', *, *, #108109, .T. ) ;
#115052=CARTESIAN_POINT ( 'NONE',  ( 65.34954526983784717, -3.515384427023117819, -5.621991122718144496 ) ) ;
#115053=CARTESIAN_POINT ( 'NONE',  ( -6.249999999999981348, 12.50000000000000000, 6.495190528383297135 ) ) ;
#115054=CARTESIAN_POINT ( 'NONE',  ( 2.499999999999981792, 2.500000000000000000, 4.330127018922196314 ) ) ;
#115055=CARTESIAN_POINT ( 'NONE',  ( 17.84432265422780262, -2.533187527835756736, 5.021315468709310892 ) ) ;
#115056=CONICAL_SURFACE ( 'NONE', #27321, 0.1000000000000002554, 0.003490658503988666988 ) ;
#115057=ORIENTED_EDGE ( 'NONE', *, *, #111689, .T. ) ;
#115058=ADVANCED_FACE ( 'NONE', ( #126223 ), #121943, .T. ) ;
#115059=VERTEX_POINT ( 'NONE', #96745 ) ;
#115060=EDGE_CURVE ( 'NONE', #120460, #125434, #90630, .T. ) ;
#115061=EDGE_LOOP ( 'NONE', ( #123370, #89244 ) ) ;
#115062=FACE_OUTER_BOUND ( 'NONE', #61606, .T. ) ;
#115063=LINE ( 'NONE', #84974, #5940 ) ;
#115064=LINE ( 'NONE', #37186, #50348 ) ;
#115065=FACE_BOUND ( 'NONE', #91454, .T. ) ;
#115066=DIRECTION ( 'NONE',  ( 0.000000000000000000, 0.000000000000000000, 1.000000000000000000 ) ) ;
#115067=FACE_OUTER_BOUND ( 'NONE', #40434, .T. ) ;
#115068=DIRECTION ( 'NONE',  ( 0.000000000000000000, 1.000000000000000000, 0.000000000000000000 ) ) ;
#115069=AXIS2_PLACEMENT_3D ( 'NONE', #74012, #83819, #31510 ) ;
#115070=AXIS2_PLACEMENT_3D ( 'NONE', #5120, #124908, #25393 ) ;
#115071=CARTESIAN_POINT ( 'NONE',  ( 14.14999999999989377, 12.50000000000000000, -2.792790559304616504 ) ) ;
#115073=DIRECTION ( 'NONE',  ( 0.000000000000000000, 0.000000000000000000, 1.000000000000000000 ) ) ;
#115074=ORIENTED_EDGE ( 'NONE', *, *, #8775, .F. ) ;
#115075=VECTOR ( 'NONE', #65982, 1000.000000000000000 ) ;
#115076=CARTESIAN_POINT ( 'NONE',  ( -3.749999999999991562, 2.500000000000000000, 6.595190528383296780 ) ) ;
#115077=ORIENTED_EDGE ( 'NONE', *, *, #65780, .T. ) ;
#115079=ORIENTED_EDGE ( 'NONE', *, *, #70845, .T. ) ;
#115080=ORIENTED_EDGE ( 'NONE', *, *, #104918, .T. ) ;
#115081=ORIENTED_EDGE ( 'NONE', *, *, #58667, .T. ) ;
#115082=CARTESIAN_POINT ( 'NONE',  ( 8.949999999999919353, 2.500000000000000000, 2.511473670974873507 ) ) ;
#115083=FACE_BOUND ( 'NONE', #2031, .T. ) ;
#115085=EDGE_LOOP ( 'NONE', ( #29868, #73136, #78240, #88526 ) ) ;
#115086=CARTESIAN_POINT ( 'NONE',  ( 81.97673105886440226, 3.779183627794353573, 6.223416391359812394 ) ) ;
#115087=DIRECTION ( 'NONE',  ( 0.000000000000000000, -0.9999939076577903929, 0.003490651415223739937 ) ) ;
#115088=ORIENTED_EDGE ( 'NONE', *, *, #18228, .T. ) ;
#115089=DIRECTION ( 'NONE',  ( 0.000000000000000000, 1.000000000000000000, 0.000000000000000000 ) ) ;
#115090=CARTESIAN_POINT ( 'NONE',  ( -1.450000000000035927, 12.50000000000000000, -1.818653347947326138 ) ) ;
#115091=EDGE_CURVE ( 'NONE', #74901, #67778, #28027, .T. ) ;
#115092=ORIENTED_EDGE ( 'NONE', *, *, #111637, .T. ) ;
#115093=AXIS2_PLACEMENT_3D ( 'NONE', #95074, #115992, #6642 ) ;
#115094=DIRECTION ( 'NONE',  ( 0.000000000000000000, 1.000000000000000000, 0.000000000000000000 ) ) ;
#115095=VECTOR ( 'NONE', #128725, 1000.000000000000000 ) ;
#115096=DIRECTION ( 'NONE',  ( -0.000000000000000000, 1.000000000000000000, -0.000000000000000000 ) ) ;
#115097=ADVANCED_FACE ( 'NONE', ( #67939 ), #25789, .T. ) ;
#115098=ORIENTED_EDGE ( 'NONE', *, *, #102451, .F. ) ;
#115099=DIRECTION ( 'NONE',  ( -4.274815082592931898E-19, -0.9999939076577903929, -0.003490651415223739937 ) ) ;
#115100=VECTOR ( 'NONE', #84484, 1000.000000000000000 ) ;
#115101=DIRECTION ( 'NONE',  ( 0.000000000000000000, 0.000000000000000000, -1.000000000000000000 ) ) ;
#115102=FACE_OUTER_BOUND ( 'NONE', #89416, .T. ) ;
#115103=ORIENTED_EDGE ( 'NONE', *, *, #35881, .T. ) ;
#115104=CONICAL_SURFACE ( 'NONE', #8506, 0.1000000000000002554, 0.003490658503988666988 ) ;
#115105=ADVANCED_FACE ( 'NONE', ( #117660 ), #741, .T. ) ;
#115106=ORIENTED_EDGE ( 'NONE', *, *, #51546, .F. ) ;
#115107=ADVANCED_FACE ( 'NONE', ( #48307 ), #113618, .T. ) ;
#115108=CARTESIAN_POINT ( 'NONE',  ( 8.549999999999918998, 12.50000000000000000, -1.753560074763288679 ) ) ;
#115109=ORIENTED_EDGE ( 'NONE', *, *, #107055, .T. ) ;
#115110=CARTESIAN_POINT ( 'NONE',  ( -5.850000000000022737, 2.500000000000000000, -6.595190528383302109 ) ) ;
#115111=DIRECTION ( 'NONE',  ( -0.000000000000000000, 1.000000000000000000, -0.000000000000000000 ) ) ;
#115112=VERTEX_POINT ( 'NONE', #39161 ) ;
#115113=DIRECTION ( 'NONE',  ( 0.000000000000000000, 0.000000000000000000, 1.000000000000000000 ) ) ;
#115114=LINE ( 'NONE', #124970, #110396 ) ;
#115115=FACE_OUTER_BOUND ( 'NONE', #17184, .T. ) ;
#115116=DIRECTION ( 'NONE',  ( 0.000000000000000000, 0.000000000000000000, -1.000000000000000000 ) ) ;
#115117=ADVANCED_FACE ( 'NONE', ( #66645 ), #29321, .T. ) ;
#115119=ORIENTED_EDGE ( 'NONE', *, *, #121970, .F. ) ;
#115120=ORIENTED_EDGE ( 'NONE', *, *, #50010, .T. ) ;
#115121=LINE ( 'NONE', #105978, #3497 ) ;
#115122=CARTESIAN_POINT ( 'NONE',  ( 10.39999999999991154, 12.50000000000000000, 3.637306695894644726 ) ) ;
#115123=CARTESIAN_POINT ( 'NONE',  ( -4.150000000000027889, 12.50000000000000000, -7.188010851410854052 ) ) ;
#115124=VERTEX_POINT ( 'NONE', #106574 ) ;
#115125=VERTEX_POINT ( 'NONE', #7070 ) ;
#115126=VERTEX_POINT ( 'NONE', #47033 ) ;
#115127=DIRECTION ( 'NONE',  ( -0.000000000000000000, -1.000000000000000000, -0.000000000000000000 ) ) ;
#115128=VECTOR ( 'NONE', #56901, 1000.000000000000000 ) ;
#115129=DIRECTION ( 'NONE',  ( -0.000000000000000000, 1.000000000000000000, -0.000000000000000000 ) ) ;
#115130=CONICAL_SURFACE ( 'NONE', #83849, 0.1000000000000000056, 0.003490658503988666988 ) ;
#115131=DIRECTION ( 'NONE',  ( 0.000000000000000000, -0.9999939076577903929, 0.003490651415223739937 ) ) ;
#115132=DIRECTION ( 'NONE',  ( 0.000000000000000000, 1.000000000000000000, 0.000000000000000000 ) ) ;
#115133=DIRECTION ( 'NONE',  ( 0.000000000000000000, 1.000000000000000000, 0.000000000000000000 ) ) ;
#115135=CARTESIAN_POINT ( 'NONE',  ( -7.100000000000013856, 2.500000000000000000, 3.637306695894644726 ) ) ;
#115136=CARTESIAN_POINT ( 'NONE',  ( 5.649999999999932854, 12.50000000000000000, 1.818653347947321475 ) ) ;
#115137=DIRECTION ( 'NONE',  ( 0.000000000000000000, 1.000000000000000000, 0.000000000000000000 ) ) ;
#115138=AXIS2_PLACEMENT_3D ( 'NONE', #113239, #63517, #103437 ) ;
#115139=EDGE_LOOP ( 'NONE', ( #62479, #118445, #90380, #122303 ) ) ;
#115140=EDGE_CURVE ( 'NONE', #948, #105841, #37214, .T. ) ;
#115141=DIRECTION ( 'NONE',  ( 0.000000000000000000, 0.000000000000000000, -1.000000000000000000 ) ) ;
#115142=VERTEX_POINT ( 'NONE', #29971 ) ;
#115143=ORIENTED_EDGE ( 'NONE', *, *, #96294, .F. ) ;
#115144=ADVANCED_FACE ( 'NONE', ( #59443 ), #44675, .T. ) ;
#115145=CARTESIAN_POINT ( 'NONE',  ( 5.449999999999936229, 2.500000000000000000, 6.495190528383297135 ) ) ;
#115146=CARTESIAN_POINT ( 'NONE',  ( -13.34999999999999076, 2.500000000000000000, -2.065063509461099844 ) ) ;
#115147=CARTESIAN_POINT ( 'NONE',  ( 6.449999999999931788, 2.500000000000000000, 6.148780366869520009 ) ) ;
#115148=EDGE_CURVE ( 'NONE', #68264, #47076, #60715, .T. ) ;
#115149=VECTOR ( 'NONE', #3823, 1000.000000000000000 ) ;
#115150=DIRECTION ( 'NONE',  ( 0.000000000000000000, 0.000000000000000000, 1.000000000000000000 ) ) ;
#115151=AXIS2_PLACEMENT_3D ( 'NONE', #49585, #67911, #89493 ) ;
#115152=DIRECTION ( 'NONE',  ( 0.000000000000000000, 0.000000000000000000, -1.000000000000000000 ) ) ;
#115153=CARTESIAN_POINT ( 'NONE',  ( -8.750000000000008882, 12.50000000000000000, 1.472243186433545459 ) ) ;
#115154=DIRECTION ( 'NONE',  ( 0.000000000000000000, 0.000000000000000000, 1.000000000000000000 ) ) ;
#115155=ORIENTED_EDGE ( 'NONE', *, *, #75461, .F. ) ;
#115156=CARTESIAN_POINT ( 'NONE',  ( 8.749999999999923617, 2.500000000000000000, -7.188010851410854052 ) ) ;
#115157=ADVANCED_FACE ( 'NONE', ( #50250 ), #42538, .T. ) ;
#115158=ADVANCED_FACE ( 'NONE', ( #91450 ), #13257, .T. ) ;
#115159=EDGE_CURVE ( 'NONE', #94964, #53612, #69219, .T. ) ;
#115160=CONICAL_SURFACE ( 'NONE', #4431, 0.09999999999999982514, 0.003490658503988666988 ) ;
#115161=ADVANCED_FACE ( 'NONE', ( #80993 ), #6985, .T. ) ;
#115163=ORIENTED_EDGE ( 'NONE', *, *, #31695, .T. ) ;
#115164=EDGE_LOOP ( 'NONE', ( #71434, #118470, #41283, #100440 ) ) ;
#115165=ADVANCED_FACE ( 'NONE', ( #20787 ), #38430, .T. ) ;
#115166=CIRCLE ( 'NONE', #29524, 0.1000000000000002554 ) ;
#115167=ORIENTED_EDGE ( 'NONE', *, *, #81644, .T. ) ;
#115168=ORIENTED_EDGE ( 'NONE', *, *, #93178, .F. ) ;
#115169=CARTESIAN_POINT ( 'NONE',  ( 3.949999999999942446, 12.50000000000000000, -2.511473670974877948 ) ) ;
#115170=CARTESIAN_POINT ( 'NONE',  ( -11.84999999999999787, 12.50000000000000000, -2.511473670974873951 ) ) ;
#115171=EDGE_CURVE ( 'NONE', #91471, #75085, #79695, .T. ) ;
#115172=DIRECTION ( 'NONE',  ( 0.000000000000000000, 1.000000000000000000, 0.000000000000000000 ) ) ;
#115173=CARTESIAN_POINT ( 'NONE',  ( -8.750000000000007105, 2.500000000000000000, 7.188010851410848723 ) ) ;
#115174=CARTESIAN_POINT ( 'NONE',  ( -5.400000000000019895, 2.500000000000000000, -0.5928203230275541635 ) ) ;
#115175=ORIENTED_EDGE ( 'NONE', *, *, #12200, .T. ) ;
#115176=DIRECTION ( 'NONE',  ( 0.000000000000000000, 0.000000000000000000, -1.000000000000000000 ) ) ;
#115177=DIRECTION ( 'NONE',  ( 0.000000000000000000, 1.000000000000000000, 0.000000000000000000 ) ) ;
#115178=DIRECTION ( 'NONE',  ( -0.000000000000000000, 1.000000000000000000, -0.000000000000000000 ) ) ;
#115179=EDGE_LOOP ( 'NONE', ( #86132, #122226, #26839, #16844 ) ) ;
#115180=ORIENTED_EDGE ( 'NONE', *, *, #58411, .F. ) ;
#115181=ORIENTED_EDGE ( 'NONE', *, *, #117636, .F. ) ;
#115182=AXIS2_PLACEMENT_3D ( 'NONE', #24225, #64141, #104075 ) ;
#115183=DIRECTION ( 'NONE',  ( 0.000000000000000000, -0.000000000000000000, 1.000000000000000000 ) ) ;
#115184=VECTOR ( 'NONE', #14242, 1000.000000000000000 ) ;
#115185=AXIS2_PLACEMENT_3D ( 'NONE', #106317, #4875, #86008 ) ;
#115186=DIRECTION ( 'NONE',  ( 0.000000000000000000, 0.000000000000000000, 1.000000000000000000 ) ) ;
#115187=DIRECTION ( 'NONE',  ( -0.000000000000000000, 1.000000000000000000, -0.000000000000000000 ) ) ;
#115188=AXIS2_PLACEMENT_3D ( 'NONE', #34099, #12508, #72733 ) ;
#115189=AXIS2_PLACEMENT_3D ( 'NONE', #114969, #105813, #3737 ) ;
#115190=AXIS2_PLACEMENT_3D ( 'NONE', #103741, #115455, #123369 ) ;
#115191=ORIENTED_EDGE ( 'NONE', *, *, #87515, .T. ) ;
#115192=CARTESIAN_POINT ( 'NONE',  ( 12.09999999999990550, 2.500000000000000000, 3.537306695894645081 ) ) ;
#115193=CARTESIAN_POINT ( 'NONE',  ( -10.65000000000000391, 2.500000000000000000, -1.818653347947322141 ) ) ;
#115194=DIRECTION ( 'NONE',  ( 0.000000000000000000, -0.000000000000000000, 1.000000000000000000 ) ) ;
#115196=CARTESIAN_POINT ( 'NONE',  ( 2.099999999999950351, 2.500000000000000000, 0.09999999999999772959 ) ) ;
#115197=VERTEX_POINT ( 'NONE', #10929 ) ;
#115198=DIRECTION ( 'NONE',  ( 0.000000000000000000, 1.000000000000000000, 0.000000000000000000 ) ) ;
#115200=VERTEX_POINT ( 'NONE', #50892 ) ;
#115201=VERTEX_POINT ( 'NONE', #89519 ) ;
#115202=ORIENTED_EDGE ( 'NONE', *, *, #57135, .T. ) ;
#115203=DIRECTION ( 'NONE',  ( 0.000000000000000000, -0.000000000000000000, 1.000000000000000000 ) ) ;
#115204=FACE_BOUND ( 'NONE', #127965, .T. ) ;
#115205=FACE_OUTER_BOUND ( 'NONE', #13057, .T. ) ;
#115206=DIRECTION ( 'NONE',  ( -0.000000000000000000, -1.000000000000000000, -0.000000000000000000 ) ) ;
#115207=CARTESIAN_POINT ( 'NONE',  ( -12.89999999999999325, 2.500000000000000000, 0.7928203230275536750 ) ) ;
#115208=ADVANCED_FACE ( 'NONE', ( #111739 ), #69803, .T. ) ;
#115209=EDGE_LOOP ( 'NONE', ( #125604, #32938, #42093, #29558 ) ) ;
#115210=FACE_OUTER_BOUND ( 'NONE', #94390, .T. ) ;
#115211=DIRECTION ( 'NONE',  ( -0.000000000000000000, -1.000000000000000000, -0.000000000000000000 ) ) ;
#115212=DIRECTION ( 'NONE',  ( 0.000000000000000000, 0.000000000000000000, 1.000000000000000000 ) ) ;
#115213=CARTESIAN_POINT ( 'NONE',  ( -7.100000000000013856, 2.500000000000000000, 5.022947341949748790 ) ) ;
#115214=ORIENTED_EDGE ( 'NONE', *, *, #65642, .F. ) ;
#115215=AXIS2_PLACEMENT_3D ( 'NONE', #99445, #569, #42460 ) ;
#115216=FACE_OUTER_BOUND ( 'NONE', #18422, .T. ) ;
#115217=VECTOR ( 'NONE', #80747, 1000.000000000000000 ) ;
#115218=CARTESIAN_POINT ( 'NONE',  ( -5.200000000000025935, 2.500000000000000000, -3.983716857408426293 ) ) ;
#115219=ORIENTED_EDGE ( 'NONE', *, *, #50196, .F. ) ;
#115220=PLANE ( 'NONE',  #41868 ) ;
#115221=EDGE_LOOP ( 'NONE', ( #117694, #42939, #108008, #47467 ) ) ;
#115222=FACE_BOUND ( 'NONE', #116914, .T. ) ;
#115223=DIRECTION ( 'NONE',  ( 0.000000000000000000, -0.9999939076577903929, 0.003490651415223739937 ) ) ;
#115225=VERTEX_POINT ( 'NONE', #119615 ) ;
#115226=DIRECTION ( 'NONE',  ( 0.000000000000000000, 0.000000000000000000, 1.000000000000000000 ) ) ;
#115227=CARTESIAN_POINT ( 'NONE',  ( 2.899999999999944844, 2.500000000000000000, 3.537306695894645081 ) ) ;
#115228=ORIENTED_EDGE ( 'NONE', *, *, #66677, .F. ) ;
#115229=ORIENTED_EDGE ( 'NONE', *, *, #102393, .F. ) ;
#115231=VERTEX_POINT ( 'NONE', #69886 ) ;
#115232=VECTOR ( 'NONE', #69835, 1000.000000000000000 ) ;
#115234=DIRECTION ( 'NONE',  ( 0.000000000000000000, 0.000000000000000000, 1.000000000000000000 ) ) ;
#115235=CIRCLE ( 'NONE', #102655, 0.06509327318403745899 ) ;
#115236=EDGE_CURVE ( 'NONE', #9888, #80502, #109809, .T. ) ;
#115237=DIRECTION ( 'NONE',  ( -4.274815082592931898E-19, -0.9999939076577903929, -0.003490651415223739937 ) ) ;
#115238=VECTOR ( 'NONE', #28616, 1000.000000000000000 ) ;
#115239=FACE_OUTER_BOUND ( 'NONE', #120181, .T. ) ;
#115240=CARTESIAN_POINT ( 'NONE',  ( -9.999999999999969802, 2.500000000000000000, 4.430127018922196847 ) ) ;
#115241=AXIS2_PLACEMENT_3D ( 'NONE', #105092, #5595, #6238 ) ;
#115242=ADVANCED_FACE ( 'NONE', ( #30622 ), #32266, .T. ) ;
#115243=ORIENTED_EDGE ( 'NONE', *, *, #104113, .T. ) ;
#115244=ORIENTED_EDGE ( 'NONE', *, *, #47334, .F. ) ;
#115245=DIRECTION ( 'NONE',  ( -4.274815082592931898E-19, -0.9999939076577903929, -0.003490651415223739937 ) ) ;
#115246=VECTOR ( 'NONE', #93076, 1000.000000000000000 ) ;
#115247=AXIS2_PLACEMENT_3D ( 'NONE', #48206, #8909, #86170 ) ;
#115248=DIRECTION ( 'NONE',  ( 0.000000000000000000, 0.000000000000000000, -1.000000000000000000 ) ) ;
#115249=DIRECTION ( 'NONE',  ( -0.000000000000000000, 1.000000000000000000, -0.000000000000000000 ) ) ;
#115250=CARTESIAN_POINT ( 'NONE',  ( 11.84999999999990372, 12.50000000000000000, -6.841600689897078702 ) ) ;
#115251=ORIENTED_EDGE ( 'NONE', *, *, #86845, .T. ) ;
#115252=VERTEX_POINT ( 'NONE', #90809 ) ;
#115253=EDGE_CURVE ( 'NONE', #4247, #28898, #41093, .T. ) ;
#115254=FACE_BOUND ( 'NONE', #49739, .T. ) ;
#115255=ORIENTED_EDGE ( 'NONE', *, *, #93928, .T. ) ;
#115256=EDGE_CURVE ( 'NONE', #11947, #64157, #48979, .T. ) ;
#115257=DIRECTION ( 'NONE',  ( 0.000000000000000000, 0.000000000000000000, 1.000000000000000000 ) ) ;
#115258=DIRECTION ( 'NONE',  ( -0.000000000000000000, -1.000000000000000000, -0.000000000000000000 ) ) ;
#115259=ORIENTED_EDGE ( 'NONE', *, *, #102696, .F. ) ;
#115260=DIRECTION ( 'NONE',  ( 0.000000000000000000, -0.000000000000000000, 1.000000000000000000 ) ) ;
#115261=CARTESIAN_POINT ( 'NONE',  ( -10.40000000000000213, 2.500000000000000000, 3.637306695894644726 ) ) ;
#115262=CARTESIAN_POINT ( 'NONE',  ( 7.499999999999925393, 2.500000000000000000, -3.737306695894649700 ) ) ;
#115263=CARTESIAN_POINT ( 'NONE',  ( 12.89999999999990266, 2.500000000000000000, 3.537306695894645081 ) ) ;
#115264=EDGE_CURVE ( 'NONE', #116433, #74234, #65591, .T. ) ;
#115268=DIRECTION ( 'NONE',  ( -0.000000000000000000, -1.000000000000000000, -0.000000000000000000 ) ) ;
#115269=ADVANCED_FACE ( 'NONE', ( #69653 ), #57278, .T. ) ;
#115270=DIRECTION ( 'NONE',  ( -0.000000000000000000, 1.000000000000000000, -0.000000000000000000 ) ) ;
#115271=VERTEX_POINT ( 'NONE', #78857 ) ;
#115272=ORIENTED_EDGE ( 'NONE', *, *, #122252, .T. ) ;
#115273=CARTESIAN_POINT ( 'NONE',  ( -0.6000000000000383915, 2.500000000000000000, -4.676537180435977881 ) ) ;
#115274=ORIENTED_EDGE ( 'NONE', *, *, #11097, .T. ) ;
#115275=CIRCLE ( 'NONE', #94455, 0.06509327318403745899 ) ;
#115276=CARTESIAN_POINT ( 'NONE',  ( 7.899999999999924860, 12.50000000000000000, 5.022947341949748790 ) ) ;
#115277=VECTOR ( 'NONE', #31818, 1000.000000000000000 ) ;
#115278=AXIS2_PLACEMENT_3D ( 'NONE', #108734, #17773, #77991 ) ;
#115279=EDGE_LOOP ( 'NONE', ( #119979, #56370 ) ) ;
#115281=ORIENTED_EDGE ( 'NONE', *, *, #47899, .T. ) ;
#115282=CARTESIAN_POINT ( 'NONE',  ( -4.150000000000025224, 2.500000000000000000, 6.495190528383297135 ) ) ;
#115283=CONICAL_SURFACE ( 'NONE', #10827, 0.09999999999999982514, 0.003490658503988666988 ) ;
#115284=CARTESIAN_POINT ( 'NONE',  ( 6.649999999999928413, 12.50000000000000000, 2.857883832488649301 ) ) ;
#115285=AXIS2_PLACEMENT_3D ( 'NONE', #18716, #49492, #87447 ) ;
#115287=LINE ( 'NONE', #15818, #47294 ) ;
#115288=CARTESIAN_POINT ( 'NONE',  ( -11.84999999999999609, 2.500000000000000000, 2.511473670974873507 ) ) ;
#115289=AXIS2_PLACEMENT_3D ( 'NONE', #37707, #27880, #67801 ) ;
#115291=ORIENTED_EDGE ( 'NONE', *, *, #116470, .F. ) ;
#115292=CARTESIAN_POINT ( 'NONE',  ( -6.650000000000015454, 2.500000000000000000, 2.757883832488649656 ) ) ;
#115293=AXIS2_PLACEMENT_3D ( 'NONE', #95955, #43653, #83574 ) ;
#115294=ORIENTED_EDGE ( 'NONE', *, *, #60971, .F. ) ;
#115295=ORIENTED_EDGE ( 'NONE', *, *, #28056, .F. ) ;
#115296=VERTEX_POINT ( 'NONE', #8147 ) ;
#115297=VERTEX_POINT ( 'NONE', #57265 ) ;
#115298=CARTESIAN_POINT ( 'NONE',  ( -0.8000000000000315747, 2.500000000000000000, 0.000000000000000000 ) ) ;
#115299=ORIENTED_EDGE ( 'NONE', *, *, #94102, .T. ) ;
#115300=VERTEX_POINT ( 'NONE', #9455 ) ;
#115301=FACE_OUTER_BOUND ( 'NONE', #68284, .T. ) ;
#115303=DIRECTION ( 'NONE',  ( -0.000000000000000000, 1.000000000000000000, -0.000000000000000000 ) ) ;
#115304=CARTESIAN_POINT ( 'NONE',  ( 2.049999999999950084, 12.50000000000000000, -6.495190528383302464 ) ) ;
#115305=FACE_OUTER_BOUND ( 'NONE', #20652, .T. ) ;
#115306=EDGE_CURVE ( 'NONE', #111256, #109372, #106986, .T. ) ;
#115307=FACE_OUTER_BOUND ( 'NONE', #100863, .T. ) ;
#115308=EDGE_LOOP ( 'NONE', ( #102558, #127293, #123723, #99003 ) ) ;
#115309=EDGE_CURVE ( 'NONE', #54837, #123253, #87985, .T. ) ;
#115310=EDGE_CURVE ( 'NONE', #122488, #37002, #59360, .T. ) ;
#115311=FACE_OUTER_BOUND ( 'NONE', #119654, .T. ) ;
#115312=ADVANCED_FACE ( 'NONE', ( #17971 ), #2906, .T. ) ;
#115313=AXIS2_PLACEMENT_3D ( 'NONE', #69305, #109232, #101369 ) ;
#115314=AXIS2_PLACEMENT_3D ( 'NONE', #9264, #28260, #100221 ) ;
#115315=EDGE_LOOP ( 'NONE', ( #117012, #43035 ) ) ;
#115316=CARTESIAN_POINT ( 'NONE',  ( -3.350000000000028511, 12.50000000000000000, -2.792790559304616504 ) ) ;
#115317=ORIENTED_EDGE ( 'NONE', *, *, #99876, .F. ) ;
#115318=CARTESIAN_POINT ( 'NONE',  ( -4.150000000000025224, 12.50000000000000000, 2.857883832488649301 ) ) ;
#115319=ADVANCED_FACE ( 'NONE', ( #108288 ), #61502, .T. ) ;
#115320=ORIENTED_EDGE ( 'NONE', *, *, #31233, .T. ) ;
#115321=EDGE_LOOP ( 'NONE', ( #34368, #103575 ) ) ;
#115322=CONICAL_SURFACE ( 'NONE', #121697, 0.1000000000000002554, 0.003490658503988666988 ) ;
#115323=CARTESIAN_POINT ( 'NONE',  ( 10.44999999999991402, 12.50000000000000000, 6.560283801567334372 ) ) ;
#115324=DIRECTION ( 'NONE',  ( 0.000000000000000000, 0.000000000000000000, 1.000000000000000000 ) ) ;
#115325=CONICAL_SURFACE ( 'NONE', #44338, 0.1000000000000000472, 0.003490658503988666988 ) ;
#115326=EDGE_CURVE ( 'NONE', #36772, #121481, #9159, .T. ) ;
#115327=VECTOR ( 'NONE', #87171, 1000.000000000000000 ) ;
#115328=ADVANCED_FACE ( 'NONE', ( #96515 ), #37635, .T. ) ;
#115329=CARTESIAN_POINT ( 'NONE',  ( 12.29999999999990301, 12.50000000000000000, -0.3464101615137782364 ) ) ;
#115330=AXIS2_PLACEMENT_3D ( 'NONE', #97973, #86862, #8938 ) ;
#115332=CARTESIAN_POINT ( 'NONE',  ( 1.649999999999948841, 2.500000000000000000, 6.495190528383297135 ) ) ;
#115333=CARTESIAN_POINT ( 'NONE',  ( -10.40000000000000213, 12.50000000000000000, 0.06509327318403515528 ) ) ;
#115334=EDGE_LOOP ( 'NONE', ( #67804, #9772 ) ) ;
#115335=DIRECTION ( 'NONE',  ( 0.000000000000000000, 1.000000000000000000, 0.000000000000000000 ) ) ;
#115336=FACE_OUTER_BOUND ( 'NONE', #52882, .T. ) ;
#115337=CARTESIAN_POINT ( 'NONE',  ( 4.399999999999940847, 2.500000000000000000, -4.776537180435977525 ) ) ;
#115338=DIRECTION ( 'NONE',  ( 0.000000000000000000, 0.000000000000000000, -1.000000000000000000 ) ) ;
#115340=AXIS2_PLACEMENT_3D ( 'NONE', #108164, #66311, #58448 ) ;
#115341=FACE_OUTER_BOUND ( 'NONE', #117491, .T. ) ;
#115342=ORIENTED_EDGE ( 'NONE', *, *, #100296, .F. ) ;
#115344=CIRCLE ( 'NONE', #46403, 0.1000000000000000056 ) ;
#115345=AXIS2_PLACEMENT_3D ( 'NONE', #105798, #63290, #92766 ) ;
#115346=VERTEX_POINT ( 'NONE', #46804 ) ;
#115347=CIRCLE ( 'NONE', #40071, 0.1000000000000002554 ) ;
#115348=ORIENTED_EDGE ( 'NONE', *, *, #65088, .T. ) ;
#115349=DIRECTION ( 'NONE',  ( -4.274815082592931898E-19, -0.9999939076577903929, -0.003490651415223739937 ) ) ;
#115350=DIRECTION ( 'NONE',  ( 0.000000000000000000, 0.000000000000000000, 1.000000000000000000 ) ) ;
#115352=DIRECTION ( 'NONE',  ( 0.000000000000000000, -0.000000000000000000, 1.000000000000000000 ) ) ;
#115353=DIRECTION ( 'NONE',  ( -0.000000000000000000, 1.000000000000000000, -0.000000000000000000 ) ) ;
#115354=DIRECTION ( 'NONE',  ( 0.000000000000000000, 0.000000000000000000, 1.000000000000000000 ) ) ;
#115355=DIRECTION ( 'NONE',  ( 0.000000000000000000, 0.000000000000000000, 1.000000000000000000 ) ) ;
#115356=ORIENTED_EDGE ( 'NONE', *, *, #53163, .T. ) ;
#115357=DIRECTION ( 'NONE',  ( -4.274815082592931898E-19, -0.9999939076577903929, -0.003490651415223739937 ) ) ;
#115358=CARTESIAN_POINT ( 'NONE',  ( -13.34999999999999076, 2.500000000000000000, -2.857883832488651521 ) ) ;
#115359=EDGE_LOOP ( 'NONE', ( #79063, #53062 ) ) ;
#115361=CARTESIAN_POINT ( 'NONE',  ( 14.54999999999989591, 2.500000000000000000, 2.165063509461097713 ) ) ;
#115362=CARTESIAN_POINT ( 'NONE',  ( 14.34999999999989306, 12.50000000000000000, -1.818653347947326138 ) ) ;
#115363=EDGE_CURVE ( 'NONE', #92822, #13065, #53078, .T. ) ;
#115364=ORIENTED_EDGE ( 'NONE', *, *, #115766, .T. ) ;
#115365=CARTESIAN_POINT ( 'NONE',  ( 3.349999999999944578, 12.50000000000000000, -1.472243186433550122 ) ) ;
#115366=CONICAL_SURFACE ( 'NONE', #21396, 0.1000000000000000472, 0.003490658503988666988 ) ;
#115367=AXIS2_PLACEMENT_3D ( 'NONE', #97681, #45380, #66919 ) ;
#115368=CONICAL_SURFACE ( 'NONE', #23459, 0.1000000000000002554, 0.003490658503988666988 ) ;
#115369=EDGE_LOOP ( 'NONE', ( #24894, #90111 ) ) ;
#115370=DIRECTION ( 'NONE',  ( 0.000000000000000000, 0.000000000000000000, 1.000000000000000000 ) ) ;
#115371=DIRECTION ( 'NONE',  ( -0.000000000000000000, 1.000000000000000000, -0.000000000000000000 ) ) ;
#115372=EDGE_LOOP ( 'NONE', ( #2947, #116738, #14972, #109754 ) ) ;
#115373=AXIS2_PLACEMENT_3D ( 'NONE', #13967, #53910, #72907 ) ;
#115374=PLANE ( 'NONE',  #105368 ) ;
#115375=AXIS2_PLACEMENT_3D ( 'NONE', #56905, #7816, #66094 ) ;
#115376=AXIS2_PLACEMENT_3D ( 'NONE', #89398, #8245, #39040 ) ;
#115377=DIRECTION ( 'NONE',  ( 0.000000000000000000, 0.000000000000000000, -1.000000000000000000 ) ) ;
#115378=AXIS2_PLACEMENT_3D ( 'NONE', #38877, #117362, #118680 ) ;
#115379=AXIS2_PLACEMENT_3D ( 'NONE', #23141, #123280, #42143 ) ;
#115380=VERTEX_POINT ( 'NONE', #77534 ) ;
#115381=CONICAL_SURFACE ( 'NONE', #90363, 0.09999999999999982514, 0.003490658503988666988 ) ;
#115382=DIRECTION ( 'NONE',  ( -0.000000000000000000, 1.000000000000000000, -0.000000000000000000 ) ) ;
#115383=ORIENTED_EDGE ( 'NONE', *, *, #93067, .T. ) ;
#115384=ORIENTED_EDGE ( 'NONE', *, *, #82356, .F. ) ;
#115385=FACE_OUTER_BOUND ( 'NONE', #71013, .T. ) ;
#115386=CARTESIAN_POINT ( 'NONE',  ( 9.599999999999917932, 12.50000000000000000, -2.276824562219559311E-15 ) ) ;
#115387=EDGE_LOOP ( 'NONE', ( #77019, #68892, #27168, #48781 ) ) ;
#115388=EDGE_CURVE ( 'NONE', #3164, #22492, #128612, .T. ) ;
#115389=DIRECTION ( 'NONE',  ( -4.274815082592931898E-19, -0.9999939076577903929, -0.003490651415223739937 ) ) ;
#115390=CARTESIAN_POINT ( 'NONE',  ( -8.300000000000011369, 2.500000000000000000, -2.276824562219559311E-15 ) ) ;
#115391=ORIENTED_EDGE ( 'NONE', *, *, #72991, .T. ) ;
#115392=CARTESIAN_POINT ( 'NONE',  ( -13.74999999999998934, 12.50000000000000000, -1.472243186433547901 ) ) ;
#115393=CARTESIAN_POINT ( 'NONE',  ( 11.04999999999990656, 2.500000000000000000, 2.611473670974873151 ) ) ;
#115394=DIRECTION ( 'NONE',  ( 0.000000000000000000, 1.000000000000000000, 0.000000000000000000 ) ) ;
#115395=LINE ( 'NONE', #25112, #50872 ) ;
#115396=CARTESIAN_POINT ( 'NONE',  ( -13.09999999999999076, 2.500000000000000000, 4.676537180435972552 ) ) ;
#115398=AXIS2_PLACEMENT_3D ( 'NONE', #3646, #62583, #63863 ) ;
#115399=EDGE_CURVE ( 'NONE', #39135, #113969, #82333, .T. ) ;
#115400=ORIENTED_EDGE ( 'NONE', *, *, #18974, .F. ) ;
#115401=ORIENTED_EDGE ( 'NONE', *, *, #94095, .F. ) ;
#115402=ORIENTED_EDGE ( 'NONE', *, *, #62445, .T. ) ;
#115403=ORIENTED_EDGE ( 'NONE', *, *, #128649, .T. ) ;
#115404=CARTESIAN_POINT ( 'NONE',  ( 11.04999999999990834, 2.500000000000000000, -6.941600689897077459 ) ) ;
#115405=CARTESIAN_POINT ( 'NONE',  ( -4.200000000000025935, 2.500000000000000000, 0.09999999999999761857 ) ) ;
#115406=CARTESIAN_POINT ( 'NONE',  ( -5.400000000000019895, 2.500000000000000000, -0.5928203230275541635 ) ) ;
#115407=ORIENTED_EDGE ( 'NONE', *, *, #111064, .F. ) ;
#115408=EDGE_CURVE ( 'NONE', #62336, #21966, #17300, .T. ) ;
#115409=FACE_BOUND ( 'NONE', #43114, .T. ) ;
#115410=VECTOR ( 'NONE', #12824, 1000.000000000000000 ) ;
#115411=EDGE_CURVE ( 'NONE', #91335, #115443, #71964, .T. ) ;
#115412=DIRECTION ( 'NONE',  ( 0.000000000000000000, -0.9999939076577903929, 0.003490651415223739937 ) ) ;
#115413=LINE ( 'NONE', #17209, #35450 ) ;
#115414=AXIS2_PLACEMENT_3D ( 'NONE', #17930, #48693, #19201 ) ;
#115415=CONICAL_SURFACE ( 'NONE', #8816, 0.1000000000000002554, 0.003490658503988666988 ) ;
#115416=DIRECTION ( 'NONE',  ( 0.000000000000000000, 0.000000000000000000, 1.000000000000000000 ) ) ;
#115417=AXIS2_PLACEMENT_3D ( 'NONE', #103780, #44874, #54656 ) ;
#115418=DIRECTION ( 'NONE',  ( 0.000000000000000000, 0.000000000000000000, -1.000000000000000000 ) ) ;
#115419=CARTESIAN_POINT ( 'NONE',  ( 7.499999999999925393, 2.500000000000000000, 5.122947341949749323 ) ) ;
#115421=DIRECTION ( 'NONE',  ( 0.000000000000000000, 0.000000000000000000, 1.000000000000000000 ) ) ;
#115422=EDGE_CURVE ( 'NONE', #79598, #9494, #25882, .T. ) ;
#115423=CARTESIAN_POINT ( 'NONE',  ( 1.649999999999951505, 2.500000000000000000, -1.472243186433550122 ) ) ;
#115424=CARTESIAN_POINT ( 'NONE',  ( 3.749999999999975131, 2.500000000000000000, 6.595190528383296780 ) ) ;
#115426=DIRECTION ( 'NONE',  ( -0.000000000000000000, -1.000000000000000000, -0.000000000000000000 ) ) ;
#115427=EDGE_CURVE ( 'NONE', #18575, #49224, #92796, .T. ) ;
#115428=EDGE_CURVE ( 'NONE', #106677, #14404, #88670, .T. ) ;
#115429=DIRECTION ( 'NONE',  ( -0.000000000000000000, -1.000000000000000000, -0.000000000000000000 ) ) ;
#115430=VECTOR ( 'NONE', #54403, 1000.000000000000000 ) ;
#115431=ORIENTED_EDGE ( 'NONE', *, *, #541, .F. ) ;
#115432=ORIENTED_EDGE ( 'NONE', *, *, #17478, .T. ) ;
#115433=ORIENTED_EDGE ( 'NONE', *, *, #110417, .F. ) ;
#115434=VECTOR ( 'NONE', #28733, 1000.000000000000000 ) ;
#115435=ORIENTED_EDGE ( 'NONE', *, *, #25517, .F. ) ;
#115436=AXIS2_PLACEMENT_3D ( 'NONE', #95544, #73306, #4540 ) ;
#115437=AXIS2_PLACEMENT_3D ( 'NONE', #122558, #13870, #44000 ) ;
#115438=DIRECTION ( 'NONE',  ( 0.000000000000000000, 0.000000000000000000, -1.000000000000000000 ) ) ;
#115439=EDGE_LOOP ( 'NONE', ( #64030, #100649 ) ) ;
#115440=DIRECTION ( 'NONE',  ( -0.000000000000000000, 1.000000000000000000, -0.000000000000000000 ) ) ;
#115441=ORIENTED_EDGE ( 'NONE', *, *, #74111, .T. ) ;
#115442=EDGE_CURVE ( 'NONE', #10889, #104716, #22515, .T. ) ;
#115443=VERTEX_POINT ( 'NONE', #42809 ) ;
#115444=AXIS2_PLACEMENT_3D ( 'NONE', #127029, #33644, #97546 ) ;
#115445=CARTESIAN_POINT ( 'NONE',  ( 0.5999999999999547917, 12.50000000000000000, 3.983716857408420076 ) ) ;
#115446=AXIS2_PLACEMENT_3D ( 'NONE', #100158, #50397, #123636 ) ;
#115447=CARTESIAN_POINT ( 'NONE',  ( 0.1999999999999567124, 2.500000000000000000, -3.883716857408426648 ) ) ;
#115449=CARTESIAN_POINT ( 'NONE',  ( -2.700000000000029932, 2.500000000000000000, -0.2464101615137782308 ) ) ;
#115450=DIRECTION ( 'NONE',  ( -4.274815082592931898E-19, -0.9999939076577903929, -0.003490651415223739937 ) ) ;
#115451=EDGE_LOOP ( 'NONE', ( #71831, #12497 ) ) ;
#115452=ORIENTED_EDGE ( 'NONE', *, *, #54434, .T. ) ;
#115453=ORIENTED_EDGE ( 'NONE', *, *, #117137, .T. ) ;
#115454=EDGE_LOOP ( 'NONE', ( #114519, #69620 ) ) ;
#115455=DIRECTION ( 'NONE',  ( -0.000000000000000000, -1.000000000000000000, -0.000000000000000000 ) ) ;
#115456=CIRCLE ( 'NONE', #7081, 0.06509327318403745899 ) ;
#115457=ORIENTED_EDGE ( 'NONE', *, *, #59026, .F. ) ;
#115458=ORIENTED_EDGE ( 'NONE', *, *, #124328, .T. ) ;
#115459=CARTESIAN_POINT ( 'NONE',  ( -9.350000000000006750, 2.500000000000000000, -2.611473670974877592 ) ) ;
#115461=LINE ( 'NONE', #75555, #62537 ) ;
#115462=VECTOR ( 'NONE', #94483, 1000.000000000000000 ) ;
#115463=CARTESIAN_POINT ( 'NONE',  ( -8.350000000000012079, 12.50000000000000000, 1.472243186433545459 ) ) ;
#115464=CIRCLE ( 'NONE', #31874, 0.1000000000000002554 ) ;
#115465=VECTOR ( 'NONE', #103441, 1000.000000000000000 ) ;
#115466=CARTESIAN_POINT ( 'NONE',  ( -11.64999999999999680, 12.50000000000000000, 5.802370205355744659 ) ) ;
#115467=CARTESIAN_POINT ( 'NONE',  ( -5.650000000000023448, 2.500000000000000000, -1.918653347947326004 ) ) ;
#115468=ADVANCED_FACE ( 'NONE', ( #122630 ), #10094, .T. ) ;
#115469=EDGE_LOOP ( 'NONE', ( #4410, #59881 ) ) ;
#115470=ADVANCED_FACE ( 'NONE', ( #51333 ), #50048, .T. ) ;
#115471=CARTESIAN_POINT ( 'NONE',  ( 4.149999999999941735, 2.500000000000000000, -7.088010851410853519 ) ) ;
#115472=VECTOR ( 'NONE', #4545, 1000.000000000000000 ) ;
#115473=AXIS2_PLACEMENT_3D ( 'NONE', #58237, #39253, #49061 ) ;
#115474=ORIENTED_EDGE ( 'NONE', *, *, #34554, .T. ) ;
#115475=CARTESIAN_POINT ( 'NONE',  ( -0.8500000000000386136, 2.500000000000000000, 5.802370205355744659 ) ) ;
#115476=ADVANCED_FACE ( 'NONE', ( #72255 ), #113718, .T. ) ;
#115477=CONICAL_SURFACE ( 'NONE', #23472, 0.09999999999999982514, 0.003490658503988666988 ) ;
#115478=ORIENTED_EDGE ( 'NONE', *, *, #80608, .T. ) ;
#115479=DIRECTION ( 'NONE',  ( 0.000000000000000000, 1.000000000000000000, 0.000000000000000000 ) ) ;
#115480=FACE_OUTER_BOUND ( 'NONE', #103999, .T. ) ;
#115481=AXIS2_PLACEMENT_3D ( 'NONE', #126259, #117059, #113372 ) ;
#115482=EDGE_LOOP ( 'NONE', ( #122857, #25105, #14328, #20534 ) ) ;
#115483=AXIS2_PLACEMENT_3D ( 'NONE', #78485, #118378, #28729 ) ;
#115484=DIRECTION ( 'NONE',  ( -0.000000000000000000, 1.000000000000000000, -0.000000000000000000 ) ) ;
#115485=EDGE_CURVE ( 'NONE', #70366, #93927, #32976, .T. ) ;
#115486=PLANE ( 'NONE',  #22787 ) ;
#115487=EDGE_LOOP ( 'NONE', ( #63206, #87385, #27455, #60055 ) ) ;
#115488=AXIS2_PLACEMENT_3D ( 'NONE', #59357, #67182, #109051 ) ;
#115489=EDGE_CURVE ( 'NONE', #69025, #90022, #102351, .T. ) ;
#115490=DIRECTION ( 'NONE',  ( -0.000000000000000000, -1.000000000000000000, -0.000000000000000000 ) ) ;
#115491=ADVANCED_FACE ( 'NONE', ( #2191 ), #257, .T. ) ;
#115492=ADVANCED_FACE ( 'NONE', ( #89933 ), #30111, .T. ) ;
#115493=CARTESIAN_POINT ( 'NONE',  ( 13.29999999999990301, 12.50000000000000000, -4.330127018922201643 ) ) ;
#115494=ORIENTED_EDGE ( 'NONE', *, *, #92577, .T. ) ;
#115495=ORIENTED_EDGE ( 'NONE', *, *, #84163, .T. ) ;
#115497=CARTESIAN_POINT ( 'NONE',  ( 6.849999999999927702, 12.50000000000000000, 1.818653347947321475 ) ) ;
#115500=EDGE_CURVE ( 'NONE', #52365, #96763, #107451, .T. ) ;
#115501=AXIS2_PLACEMENT_3D ( 'NONE', #19268, #940, #40893 ) ;
#115502=DIRECTION ( 'NONE',  ( 0.000000000000000000, 0.000000000000000000, 1.000000000000000000 ) ) ;
#115503=CARTESIAN_POINT ( 'NONE',  ( -1.650000000000034328, 2.500000000000000000, -7.088010851410853519 ) ) ;
#115504=AXIS2_PLACEMENT_3D ( 'NONE', #7506, #15378, #46805 ) ;
#115505=ORIENTED_EDGE ( 'NONE', *, *, #17863, .T. ) ;
#115506=AXIS2_PLACEMENT_3D ( 'NONE', #55381, #27196, #26566 ) ;
#115507=CARTESIAN_POINT ( 'NONE',  ( -8.550000000000007816, 2.500000000000000000, 6.248780366869520542 ) ) ;
#115508=AXIS2_PLACEMENT_3D ( 'NONE', #44613, #55076, #96268 ) ;
#115509=ORIENTED_EDGE ( 'NONE', *, *, #76204, .T. ) ;
#115510=PLANE ( 'NONE',  #7832 ) ;
#115511=EDGE_CURVE ( 'NONE', #37234, #38808, #82047, .T. ) ;
#115512=DIRECTION ( 'NONE',  ( -0.000000000000000000, -1.000000000000000000, -0.000000000000000000 ) ) ;
#115513=CARTESIAN_POINT ( 'NONE',  ( -3.749999999999991562, 12.50000000000000000, 6.495190528383297135 ) ) ;
#115514=CIRCLE ( 'NONE', #42293, 0.1000000000000002554 ) ;
#115515=AXIS2_PLACEMENT_3D ( 'NONE', #18259, #58837, #45966 ) ;
#115516=EDGE_LOOP ( 'NONE', ( #123212, #45958 ) ) ;
#115517=CIRCLE ( 'NONE', #109168, 0.1000000000000002554 ) ;
#115518=CIRCLE ( 'NONE', #123845, 0.06509327318403745899 ) ;
#115519=CARTESIAN_POINT ( 'NONE',  ( 3.099999999999943245, 12.50000000000000000, 4.048810130592458201 ) ) ;
#115520=CARTESIAN_POINT ( 'NONE',  ( -3.550000000000027356, 2.500000000000000000, -2.611473670974877592 ) ) ;
#115521=AXIS2_PLACEMENT_3D ( 'NONE', #95603, #5906, #49101 ) ;
#115522=ORIENTED_EDGE ( 'NONE', *, *, #44030, .T. ) ;
#115523=PLANE ( 'NONE',  #32216 ) ;
#115524=AXIS2_PLACEMENT_3D ( 'NONE', #108661, #10460, #68740 ) ;
#115525=EDGE_CURVE ( 'NONE', #67710, #104178, #103254, .T. ) ;
#115526=EDGE_LOOP ( 'NONE', ( #75928, #121548 ) ) ;
#115527=AXIS2_PLACEMENT_3D ( 'NONE', #59505, #99407, #70578 ) ;
#115528=VECTOR ( 'NONE', #3620, 1000.000000000000000 ) ;
#115529=VERTEX_POINT ( 'NONE', #52591 ) ;
#115530=AXIS2_PLACEMENT_3D ( 'NONE', #13051, #60889, #100797 ) ;
#115531=CARTESIAN_POINT ( 'NONE',  ( 14.39999999999989555, 12.50000000000000000, -0.3464101615137782364 ) ) ;
#115532=AXIS2_PLACEMENT_3D ( 'NONE', #74539, #65345, #37834 ) ;
#115533=EDGE_LOOP ( 'NONE', ( #56599, #23680 ) ) ;
#115534=CARTESIAN_POINT ( 'NONE',  ( -13.74999999999998757, 12.50000000000000000, 1.537336459617586915 ) ) ;
#115535=CARTESIAN_POINT ( 'NONE',  ( -0.8500000000000395017, 12.50000000000000000, 6.430097255199259010 ) ) ;
#115536=DIRECTION ( 'NONE',  ( 0.000000000000000000, 1.000000000000000000, 0.000000000000000000 ) ) ;
#115537=ORIENTED_EDGE ( 'NONE', *, *, #63871, .F. ) ;
#115538=FACE_BOUND ( 'NONE', #11946, .T. ) ;
#115539=DIRECTION ( 'NONE',  ( -0.000000000000000000, 1.000000000000000000, -0.000000000000000000 ) ) ;
#115540=ORIENTED_EDGE ( 'NONE', *, *, #97026, .F. ) ;
#115541=LINE ( 'NONE', #63888, #29761 ) ;
#115542=EDGE_CURVE ( 'NONE', #86677, #46500, #30406, .T. ) ;
#115543=CARTESIAN_POINT ( 'NONE',  ( -0.2000000000000347888, 2.500000000000000000, 0.4464101615137758272 ) ) ;
#115544=ORIENTED_EDGE ( 'NONE', *, *, #83711, .F. ) ;
#115545=EDGE_LOOP ( 'NONE', ( #73564, #105849, #61834, #40883 ) ) ;
#115546=ORIENTED_EDGE ( 'NONE', *, *, #110600, .T. ) ;
#115547=DIRECTION ( 'NONE',  ( -0.000000000000000000, -1.000000000000000000, -0.000000000000000000 ) ) ;
#115548=DIRECTION ( 'NONE',  ( -0.000000000000000000, -1.000000000000000000, -0.000000000000000000 ) ) ;
#115549=CONICAL_SURFACE ( 'NONE', #67527, 0.1000000000000002554, 0.003490658503988666988 ) ;
#115550=DIRECTION ( 'NONE',  ( 0.000000000000000000, 0.000000000000000000, 1.000000000000000000 ) ) ;
#115551=AXIS2_PLACEMENT_3D ( 'NONE', #83180, #94267, #94921 ) ;
#115552=FACE_BOUND ( 'NONE', #32717, .T. ) ;
#115555=CARTESIAN_POINT ( 'NONE',  ( 97.50000000000000000, 9.184850993605147944E-16, -7.500000000000000000 ) ) ;
#115556=CARTESIAN_POINT ( 'NONE',  ( 7.099999999999928590, 12.50000000000000000, 4.330127018922196314 ) ) ;
#115557=AXIS2_PLACEMENT_3D ( 'NONE', #118930, #57438, #97354 ) ;
#115558=FACE_OUTER_BOUND ( 'NONE', #122075, .T. ) ;
#115560=AXIS2_PLACEMENT_3D ( 'NONE', #35941, #75851, #107898 ) ;
#115561=LINE ( 'NONE', #6888, #27637 ) ;
#115562=VECTOR ( 'NONE', #106964, 1000.000000000000000 ) ;
#115563=CARTESIAN_POINT ( 'NONE',  ( -6.700000000000019718, 12.50000000000000000, -4.265033745738164406 ) ) ;
#115564=DIRECTION ( 'NONE',  ( 0.000000000000000000, -0.9999939076577903929, 0.003490651415223739937 ) ) ;
#115565=CARTESIAN_POINT ( 'NONE',  ( -2.100000000000033396, 2.500000000000000000, 0.6928203230275494784 ) ) ;
#115566=CONICAL_SURFACE ( 'NONE', #17365, 0.09999999999999982514, 0.003490658503988666988 ) ;
#115567=AXIS2_PLACEMENT_3D ( 'NONE', #117595, #9605, #79014 ) ;
#115568=FACE_OUTER_BOUND ( 'NONE', #69697, .T. ) ;
#115569=CONICAL_SURFACE ( 'NONE', #94649, 0.09999999999999982514, 0.003490658503988666988 ) ;
#115570=EDGE_CURVE ( 'NONE', #77506, #70902, #15590, .T. ) ;
#115572=VERTEX_POINT ( 'NONE', #71591 ) ;
#115573=EDGE_LOOP ( 'NONE', ( #129138, #77263, #42401, #110933 ) ) ;
#115574=VERTEX_POINT ( 'NONE', #111509 ) ;
#115575=VECTOR ( 'NONE', #108551, 1000.000000000000000 ) ;
#115576=ORIENTED_EDGE ( 'NONE', *, *, #19091, .F. ) ;
#115577=DIRECTION ( 'NONE',  ( -0.000000000000000000, -1.000000000000000000, -0.000000000000000000 ) ) ;
#115578=AXIS2_PLACEMENT_3D ( 'NONE', #19534, #59501, #60759 ) ;
#115579=LINE ( 'NONE', #26579, #2783 ) ;
#115580=EDGE_LOOP ( 'NONE', ( #115683, #33611 ) ) ;
#115581=FACE_BOUND ( 'NONE', #97834, .T. ) ;
#115582=CIRCLE ( 'NONE', #124006, 0.06509327318403745899 ) ;
#115583=CARTESIAN_POINT ( 'NONE',  ( -13.09999999999999076, 12.50000000000000000, 4.676537180435972552 ) ) ;
#115584=CARTESIAN_POINT ( 'NONE',  ( -3.100000000000028511, 12.50000000000000000, -4.676537180435977881 ) ) ;
#115585=EDGE_CURVE ( 'NONE', #107896, #104107, #11393, .T. ) ;
#115586=DIRECTION ( 'NONE',  ( -0.000000000000000000, -1.000000000000000000, -0.000000000000000000 ) ) ;
#115587=EDGE_CURVE ( 'NONE', #57456, #98705, #19727, .T. ) ;
#115588=DIRECTION ( 'NONE',  ( 0.000000000000000000, 0.000000000000000000, 1.000000000000000000 ) ) ;
#115589=EDGE_CURVE ( 'NONE', #106720, #43544, #65769, .T. ) ;
#115590=FACE_OUTER_BOUND ( 'NONE', #76815, .T. ) ;
#115591=EDGE_CURVE ( 'NONE', #121302, #1776, #43442, .T. ) ;
#115592=ORIENTED_EDGE ( 'NONE', *, *, #114546, .F. ) ;
#115593=FACE_OUTER_BOUND ( 'NONE', #79179, .T. ) ;
#115594=VERTEX_POINT ( 'NONE', #125833 ) ;
#115595=ORIENTED_EDGE ( 'NONE', *, *, #108084, .T. ) ;
#115596=VERTEX_POINT ( 'NONE', #95746 ) ;
#115597=CARTESIAN_POINT ( 'NONE',  ( -4.150000000000025224, 12.50000000000000000, -1.537336459617587581 ) ) ;
#115598=DIRECTION ( 'NONE',  ( 0.000000000000000000, -0.9999939076577903929, 0.003490651415223739937 ) ) ;
#115599=FACE_OUTER_BOUND ( 'NONE', #111868, .T. ) ;
#115600=ORIENTED_EDGE ( 'NONE', *, *, #79761, .F. ) ;
#115601=ADVANCED_FACE ( 'NONE', ( #85272 ), #23936, .T. ) ;
#115602=CARTESIAN_POINT ( 'NONE',  ( 15.50772381592150850, 1.500000000000000888, -6.996973294590575598 ) ) ;
#115603=VECTOR ( 'NONE', #49081, 1000.000000000000000 ) ;
#115604=CIRCLE ( 'NONE', #27884, 0.1000000000000002554 ) ;
#115605=EDGE_CURVE ( 'NONE', #86614, #34741, #104899, .T. ) ;
#115606=CIRCLE ( 'NONE', #691, 0.1000000000000000056 ) ;
#115607=FACE_OUTER_BOUND ( 'NONE', #69928, .T. ) ;
#115608=ADVANCED_FACE ( 'NONE', ( #93182 ), #65630, .T. ) ;
#115609=DIRECTION ( 'NONE',  ( 0.000000000000000000, 0.000000000000000000, -1.000000000000000000 ) ) ;
#115611=FACE_OUTER_BOUND ( 'NONE', #100787, .T. ) ;
#115613=DIRECTION ( 'NONE',  ( -0.000000000000000000, 1.000000000000000000, -0.000000000000000000 ) ) ;
#115614=CIRCLE ( 'NONE', #27791, 0.06509327318403745899 ) ;
#115615=ORIENTED_EDGE ( 'NONE', *, *, #15703, .T. ) ;
#115616=FACE_OUTER_BOUND ( 'NONE', #44048, .T. ) ;
#115617=AXIS2_PLACEMENT_3D ( 'NONE', #108414, #117565, #58684 ) ;
#115618=AXIS2_PLACEMENT_3D ( 'NONE', #125124, #95023, #65551 ) ;
#115619=VERTEX_POINT ( 'NONE', #85904 ) ;
#115620=AXIS2_PLACEMENT_3D ( 'NONE', #15213, #65624, #125199 ) ;
#115621=VERTEX_POINT ( 'NONE', #5417 ) ;
#115622=DIRECTION ( 'NONE',  ( 0.000000000000000000, 0.000000000000000000, 1.000000000000000000 ) ) ;
#115623=DIRECTION ( 'NONE',  ( 0.000000000000000000, -0.000000000000000000, 1.000000000000000000 ) ) ;
#115624=DIRECTION ( 'NONE',  ( 0.000000000000000000, 0.000000000000000000, -1.000000000000000000 ) ) ;
#115625=CIRCLE ( 'NONE', #11069, 0.09999999999999982514 ) ;
#115626=VERTEX_POINT ( 'NONE', #103638 ) ;
#115627=ORIENTED_EDGE ( 'NONE', *, *, #53880, .F. ) ;
#115629=DIRECTION ( 'NONE',  ( -4.274815082592931898E-19, -0.9999939076577903929, -0.003490651415223739937 ) ) ;
#115630=AXIS2_PLACEMENT_3D ( 'NONE', #61155, #62460, #112189 ) ;
#115631=AXIS2_PLACEMENT_3D ( 'NONE', #128583, #47423, #118727 ) ;
#115632=CONICAL_SURFACE ( 'NONE', #2778, 0.1000000000000002554, 0.003490658503988666988 ) ;
#115633=CARTESIAN_POINT ( 'NONE',  ( -6.650000000000019007, 2.500000000000000000, -5.902370205355750521 ) ) ;
#115634=VERTEX_POINT ( 'NONE', #15222 ) ;
#115635=ORIENTED_EDGE ( 'NONE', *, *, #25797, .T. ) ;
#115636=CARTESIAN_POINT ( 'NONE',  ( -14.14999999999998614, 2.500000000000000000, 2.065063509461101621 ) ) ;
#115637=VECTOR ( 'NONE', #19475, 1000.000000000000000 ) ;
#115638=VERTEX_POINT ( 'NONE', #36195 ) ;
#115639=CARTESIAN_POINT ( 'NONE',  ( -5.600000000000023626, 12.50000000000000000, -4.611443907251939756 ) ) ;
#115640=CARTESIAN_POINT ( 'NONE',  ( -5.650000000000019895, 12.50000000000000000, 2.511473670974873507 ) ) ;
#115641=ORIENTED_EDGE ( 'NONE', *, *, #99841, .F. ) ;
#115642=AXIS2_PLACEMENT_3D ( 'NONE', #48168, #56671, #88056 ) ;
#115643=CARTESIAN_POINT ( 'NONE',  ( 5.649999999999932854, 12.50000000000000000, 2.576566944158910744 ) ) ;
#115644=DIRECTION ( 'NONE',  ( 0.000000000000000000, -0.9999939076577903929, 0.003490651415223739937 ) ) ;
#115645=CARTESIAN_POINT ( 'NONE',  ( -0.8500000000000395017, 2.500000000000000000, 6.495190528383297135 ) ) ;
#115646=PLANE ( 'NONE',  #100233 ) ;
#115647=ORIENTED_EDGE ( 'NONE', *, *, #29308, .F. ) ;
#115648=EDGE_CURVE ( 'NONE', #120245, #62516, #74816, .T. ) ;
#115649=FACE_OUTER_BOUND ( 'NONE', #85096, .T. ) ;
#115650=CARTESIAN_POINT ( 'NONE',  ( -6.071532165918824830E-15, 2.500000000000000000, -4.330127018922201643 ) ) ;
#115651=EDGE_CURVE ( 'NONE', #18238, #91316, #13947, .T. ) ;
#115652=ORIENTED_EDGE ( 'NONE', *, *, #52665, .T. ) ;
#115655=VECTOR ( 'NONE', #27889, 1000.000000000000000 ) ;
#115657=CARTESIAN_POINT ( 'NONE',  ( -13.54999999999998828, 2.500000000000000000, -2.511473670974875727 ) ) ;
#115658=CARTESIAN_POINT ( 'NONE',  ( 6.249999999999930722, 2.500000000000000000, 1.372243186433545370 ) ) ;
#115659=DIRECTION ( 'NONE',  ( 0.000000000000000000, 0.000000000000000000, -1.000000000000000000 ) ) ;
#115660=LINE ( 'NONE', #87485, #53170 ) ;
#115662=CARTESIAN_POINT ( 'NONE',  ( 11.64999999999990443, 2.500000000000000000, -5.902370205355750521 ) ) ;
#115663=CIRCLE ( 'NONE', #82229, 0.1000000000000002554 ) ;
#115664=PLANE ( 'NONE',  #19628 ) ;
#115665=CONICAL_SURFACE ( 'NONE', #63450, 0.1000000000000000472, 0.003490658503988666988 ) ;
#115666=DIRECTION ( 'NONE',  ( 0.000000000000000000, 0.000000000000000000, 1.000000000000000000 ) ) ;
#115667=CARTESIAN_POINT ( 'NONE',  ( 3.749999999999942268, 12.50000000000000000, -5.802370205355749988 ) ) ;
#115668=CONICAL_SURFACE ( 'NONE', #23753, 0.09999999999999982514, 0.003490658503988666988 ) ;
#115669=CIRCLE ( 'NONE', #46730, 0.06509327318403745899 ) ;
#115670=DIRECTION ( 'NONE',  ( -0.000000000000000000, 1.000000000000000000, -0.000000000000000000 ) ) ;
#115671=ORIENTED_EDGE ( 'NONE', *, *, #66093, .F. ) ;
#115672=AXIS2_PLACEMENT_3D ( 'NONE', #44547, #84475, #74644 ) ;
#115673=CIRCLE ( 'NONE', #63457, 0.1000000000000000472 ) ;
#115674=CIRCLE ( 'NONE', #128222, 0.06509327318403745899 ) ;
#115675=ORIENTED_EDGE ( 'NONE', *, *, #100691, .T. ) ;
#115676=CIRCLE ( 'NONE', #30027, 0.06509327318403745899 ) ;
#115677=AXIS2_PLACEMENT_3D ( 'NONE', #31480, #90373, #71375 ) ;
#115678=VERTEX_POINT ( 'NONE', #13297 ) ;
#115679=FACE_OUTER_BOUND ( 'NONE', #106915, .T. ) ;
#115680=DIRECTION ( 'NONE',  ( -0.000000000000000000, 1.000000000000000000, -0.000000000000000000 ) ) ;
#115681=CARTESIAN_POINT ( 'NONE',  ( 10.39999999999990976, 2.500000000000000000, -4.330127018922201643 ) ) ;
#115682=CIRCLE ( 'NONE', #23465, 0.09999999999999982514 ) ;
#115683=ORIENTED_EDGE ( 'NONE', *, *, #45304, .F. ) ;
#115684=CARTESIAN_POINT ( 'NONE',  ( 19.95908882845301235, -2.629614671951224114, -2.273431397254409791 ) ) ;
#115685=DIRECTION ( 'NONE',  ( 0.000000000000000000, 0.000000000000000000, -1.000000000000000000 ) ) ;
#115686=DIRECTION ( 'NONE',  ( 0.000000000000000000, -0.000000000000000000, 1.000000000000000000 ) ) ;
#115687=ORIENTED_EDGE ( 'NONE', *, *, #93150, .F. ) ;
#115688=CIRCLE ( 'NONE', #13284, 0.06509327318403745899 ) ;
#115689=CARTESIAN_POINT ( 'NONE',  ( -9.150000000000011013, 2.500000000000000000, -5.902370205355745192 ) ) ;
#115690=ORIENTED_EDGE ( 'NONE', *, *, #53732, .T. ) ;
#115691=EDGE_CURVE ( 'NONE', #10004, #127025, #105566, .T. ) ;
#115692=EDGE_LOOP ( 'NONE', ( #56603, #15874 ) ) ;
#115693=VERTEX_POINT ( 'NONE', #44064 ) ;
#115694=ORIENTED_EDGE ( 'NONE', *, *, #124345, .T. ) ;
#115695=DIRECTION ( 'NONE',  ( -4.274815082592931898E-19, -0.9999939076577903929, -0.003490651415223739937 ) ) ;
#115696=DIRECTION ( 'NONE',  ( -0.000000000000000000, 1.000000000000000000, -0.000000000000000000 ) ) ;
#115697=VECTOR ( 'NONE', #80473, 1000.000000000000000 ) ;
#115698=DIRECTION ( 'NONE',  ( 0.000000000000000000, 1.000000000000000000, 0.000000000000000000 ) ) ;
#115699=VECTOR ( 'NONE', #40099, 1000.000000000000000 ) ;
#115700=FACE_OUTER_BOUND ( 'NONE', #14478, .T. ) ;
#115701=AXIS2_PLACEMENT_3D ( 'NONE', #74351, #114271, #104453 ) ;
#115702=EDGE_LOOP ( 'NONE', ( #16212, #7519 ) ) ;
#115703=CARTESIAN_POINT ( 'NONE',  ( 11.84999999999990727, 2.500000000000000000, -1.818653347947326138 ) ) ;
#115704=EDGE_CURVE ( 'NONE', #74258, #94015, #3002, .T. ) ;
#115705=ORIENTED_EDGE ( 'NONE', *, *, #51746, .F. ) ;
#115706=CARTESIAN_POINT ( 'NONE',  ( 17.50000000000000000, 2.500000000000000000, 0.000000000000000000 ) ) ;
#115707=CARTESIAN_POINT ( 'NONE',  ( 16.31259999906291114, -2.499999999999869882, -6.357732693022873249 ) ) ;
#115708=LINE ( 'NONE', #96077, #123791 ) ;
#115709=CARTESIAN_POINT ( 'NONE',  ( 16.86689433361524237, -2.548103353433781137, 5.776876940645016667 ) ) ;
#115710=EDGE_CURVE ( 'NONE', #106656, #71464, #97079, .T. ) ;
#115711=AXIS2_PLACEMENT_3D ( 'NONE', #72604, #11737, #43799 ) ;
#115712=AXIS2_PLACEMENT_3D ( 'NONE', #112297, #90715, #80259 ) ;
#115713=AXIS2_PLACEMENT_3D ( 'NONE', #60883, #68766, #125445 ) ;
#115714=EDGE_LOOP ( 'NONE', ( #5744, #103608, #79253, #43291 ) ) ;
#115715=AXIS2_PLACEMENT_3D ( 'NONE', #59391, #66112, #39103 ) ;
#115716=VERTEX_POINT ( 'NONE', #53886 ) ;
#115717=ORIENTED_EDGE ( 'NONE', *, *, #84449, .F. ) ;
#115718=CARTESIAN_POINT ( 'NONE',  ( -2.700000000000030820, 12.50000000000000000, 0.2813168883297361700 ) ) ;
#115719=DIRECTION ( 'NONE',  ( 0.000000000000000000, 0.000000000000000000, 1.000000000000000000 ) ) ;
#115720=ADVANCED_FACE ( 'NONE', ( #93815 ), #74103, .T. ) ;
#115721=CARTESIAN_POINT ( 'NONE',  ( 1.249999999999952038, 2.500000000000000000, 2.957883832488649389 ) ) ;
#115722=FACE_BOUND ( 'NONE', #98642, .T. ) ;
#115723=DIRECTION ( 'NONE',  ( 0.000000000000000000, 0.000000000000000000, -1.000000000000000000 ) ) ;
#115724=DIRECTION ( 'NONE',  ( 0.000000000000000000, 0.000000000000000000, 1.000000000000000000 ) ) ;
#115725=CARTESIAN_POINT ( 'NONE',  ( -3.350000000000028511, 12.50000000000000000, -1.407149913249512663 ) ) ;
#115726=DIRECTION ( 'NONE',  ( -0.000000000000000000, -1.000000000000000000, -0.000000000000000000 ) ) ;
#115727=CIRCLE ( 'NONE', #119943, 0.1000000000000002554 ) ;
#115728=CONICAL_SURFACE ( 'NONE', #105275, 0.09999999999999982514, 0.003490658503988666988 ) ;
#115729=CIRCLE ( 'NONE', #59334, 0.06509327318403745899 ) ;
#115731=CARTESIAN_POINT ( 'NONE',  ( 7.099999999999927702, 12.50000000000000000, 5.088040615133786027 ) ) ;
#115732=CIRCLE ( 'NONE', #117772, 0.09999999999999982514 ) ;
#115733=CARTESIAN_POINT ( 'NONE',  ( 2.099999999999950351, 12.50000000000000000, -4.330127018922201643 ) ) ;
#115734=AXIS2_PLACEMENT_3D ( 'NONE', #84017, #15258, #123941 ) ;
#115735=DIRECTION ( 'NONE',  ( -0.000000000000000000, -1.000000000000000000, -0.000000000000000000 ) ) ;
#115736=EDGE_CURVE ( 'NONE', #61169, #91540, #123905, .T. ) ;
#115737=ORIENTED_EDGE ( 'NONE', *, *, #66565, .T. ) ;
#115738=EDGE_LOOP ( 'NONE', ( #43554, #8274 ) ) ;
#115739=ORIENTED_EDGE ( 'NONE', *, *, #66586, .T. ) ;
#115740=ORIENTED_EDGE ( 'NONE', *, *, #58889, .F. ) ;
#115741=DIRECTION ( 'NONE',  ( -0.000000000000000000, 1.000000000000000000, -0.000000000000000000 ) ) ;
#115742=FACE_BOUND ( 'NONE', #114445, .T. ) ;
#115743=DIRECTION ( 'NONE',  ( 0.000000000000000000, 1.000000000000000000, 0.000000000000000000 ) ) ;
#115744=EDGE_CURVE ( 'NONE', #90590, #93494, #74173, .T. ) ;
#115745=VECTOR ( 'NONE', #86836, 1000.000000000000000 ) ;
#115746=ORIENTED_EDGE ( 'NONE', *, *, #120603, .T. ) ;
#115747=EDGE_CURVE ( 'NONE', #110840, #24259, #4760, .T. ) ;
#115748=CARTESIAN_POINT ( 'NONE',  ( 81.97643238330996951, 3.858501987875655903, 6.173828415102756928 ) ) ;
#115749=AXIS2_PLACEMENT_3D ( 'NONE', #48322, #79087, #89534 ) ;
#115750=EDGE_CURVE ( 'NONE', #47076, #51861, #72054, .T. ) ;
#115751=CARTESIAN_POINT ( 'NONE',  ( -0.4500000000000397571, 2.500000000000000000, -2.165063509461101710 ) ) ;
#115752=EDGE_CURVE ( 'NONE', #53951, #78167, #10825, .T. ) ;
#115753=EDGE_CURVE ( 'NONE', #98217, #78977, #88766, .T. ) ;
#115754=VERTEX_POINT ( 'NONE', #21309 ) ;
#115755=CARTESIAN_POINT ( 'NONE',  ( 9.149999999999920419, 2.500000000000000000, 2.957883832488649389 ) ) ;
#115756=DIRECTION ( 'NONE',  ( 0.000000000000000000, 0.000000000000000000, 1.000000000000000000 ) ) ;
#115757=AXIS2_PLACEMENT_3D ( 'NONE', #23420, #43744, #55476 ) ;
#115758=VECTOR ( 'NONE', #58563, 1000.000000000000000 ) ;
#115759=CONICAL_SURFACE ( 'NONE', #84473, 0.1000000000000002554, 0.003490658503988666988 ) ;
#115760=ADVANCED_FACE ( 'NONE', ( #101175 ), #112289, .T. ) ;
#115761=ORIENTED_EDGE ( 'NONE', *, *, #37728, .F. ) ;
#115762=DIRECTION ( 'NONE',  ( 0.000000000000000000, 0.000000000000000000, 1.000000000000000000 ) ) ;
#115763=EDGE_CURVE ( 'NONE', #5094, #6351, #99144, .T. ) ;
#115764=CARTESIAN_POINT ( 'NONE',  ( 3.549999999999942091, 2.500000000000000000, 2.511473670974873507 ) ) ;
#115765=AXIS2_PLACEMENT_3D ( 'NONE', #43132, #50347, #31365 ) ;
#115766=EDGE_CURVE ( 'NONE', #103538, #48968, #69324, .T. ) ;
#115767=CIRCLE ( 'NONE', #80279, 0.1000000000000002554 ) ;
#115768=ORIENTED_EDGE ( 'NONE', *, *, #91526, .F. ) ;
#115769=AXIS2_PLACEMENT_3D ( 'NONE', #22557, #62480, #63758 ) ;
#115770=DIRECTION ( 'NONE',  ( 0.000000000000000000, -0.9999939076577903929, 0.003490651415223739937 ) ) ;
#115771=EDGE_CURVE ( 'NONE', #85218, #97290, #86604, .T. ) ;
#115772=CARTESIAN_POINT ( 'NONE',  ( -7.050000000000013145, 12.50000000000000000, 6.495190528383297135 ) ) ;
#115773=ORIENTED_EDGE ( 'NONE', *, *, #44067, .T. ) ;
#115774=DIRECTION ( 'NONE',  ( 0.000000000000000000, 0.000000000000000000, 1.000000000000000000 ) ) ;
#115775=AXIS2_PLACEMENT_3D ( 'NONE', #13747, #53691, #74619 ) ;
#115776=EDGE_LOOP ( 'NONE', ( #23042, #11811, #69255, #53947 ) ) ;
#115777=ORIENTED_EDGE ( 'NONE', *, *, #55873, .F. ) ;
#115778=FACE_OUTER_BOUND ( 'NONE', #40641, .T. ) ;
#115779=ADVANCED_FACE ( 'NONE', ( #33714 ), #109609, .T. ) ;
#115780=EDGE_LOOP ( 'NONE', ( #41209, #98694, #68289, #18278 ) ) ;
#115781=DIRECTION ( 'NONE',  ( -0.000000000000000000, 1.000000000000000000, -0.000000000000000000 ) ) ;
#115782=DIRECTION ( 'NONE',  ( 0.000000000000000000, 0.000000000000000000, -1.000000000000000000 ) ) ;
#115783=EDGE_LOOP ( 'NONE', ( #105116, #32240 ) ) ;
#115784=DIRECTION ( 'NONE',  ( 0.000000000000000000, 1.000000000000000000, 0.000000000000000000 ) ) ;
#115785=CARTESIAN_POINT ( 'NONE',  ( 8.749999999999923617, 2.500000000000000000, 1.472243186433545459 ) ) ;
#115786=DIRECTION ( 'NONE',  ( -4.274815082592931898E-19, -0.9999939076577903929, -0.003490651415223739937 ) ) ;
#115787=FACE_OUTER_BOUND ( 'NONE', #1042, .T. ) ;
#115788=DIRECTION ( 'NONE',  ( -0.000000000000000000, 1.000000000000000000, -0.000000000000000000 ) ) ;
#115789=CARTESIAN_POINT ( 'NONE',  ( 6.049999999999934097, 2.500000000000000000, 6.148780366869520897 ) ) ;
#115790=AXIS2_PLACEMENT_3D ( 'NONE', #10446, #18327, #98178 ) ;
#115791=ORIENTED_EDGE ( 'NONE', *, *, #52066, .T. ) ;
#115792=VERTEX_POINT ( 'NONE', #71707 ) ;
#115793=DIRECTION ( 'NONE',  ( 0.000000000000000000, 0.000000000000000000, -1.000000000000000000 ) ) ;
#115794=PLANE ( 'NONE',  #80792 ) ;
#115795=DIRECTION ( 'NONE',  ( 0.000000000000000000, 0.000000000000000000, 1.000000000000000000 ) ) ;
#115796=EDGE_LOOP ( 'NONE', ( #67292, #76898, #19503, #78747 ) ) ;
#115797=VERTEX_POINT ( 'NONE', #3612 ) ;
#115798=ORIENTED_EDGE ( 'NONE', *, *, #51059, .T. ) ;
#115799=DIRECTION ( 'NONE',  ( 0.000000000000000000, 1.000000000000000000, 0.000000000000000000 ) ) ;
#115800=VECTOR ( 'NONE', #42365, 1000.000000000000000 ) ;
#115801=DIRECTION ( 'NONE',  ( -0.000000000000000000, 1.000000000000000000, -0.000000000000000000 ) ) ;
#115802=AXIS2_PLACEMENT_3D ( 'NONE', #106078, #16375, #25563 ) ;
#115803=DIRECTION ( 'NONE',  ( -0.000000000000000000, -1.000000000000000000, -0.000000000000000000 ) ) ;
#115805=CARTESIAN_POINT ( 'NONE',  ( 0.3999999999999559464, 2.500000000000000000, -4.330127018922201643 ) ) ;
#115806=DIRECTION ( 'NONE',  ( -4.274815082592931898E-19, -0.9999939076577903929, -0.003490651415223739937 ) ) ;
#115807=DIRECTION ( 'NONE',  ( 0.000000000000000000, 0.000000000000000000, 1.000000000000000000 ) ) ;
#115808=DIRECTION ( 'NONE',  ( 0.000000000000000000, 1.000000000000000000, 0.000000000000000000 ) ) ;
#115809=DIRECTION ( 'NONE',  ( 0.000000000000000000, 1.000000000000000000, 0.000000000000000000 ) ) ;
#115810=AXIS2_PLACEMENT_3D ( 'NONE', #92066, #112371, #52795 ) ;
#115811=FACE_OUTER_BOUND ( 'NONE', #39532, .T. ) ;
#115812=AXIS2_PLACEMENT_3D ( 'NONE', #53980, #23216, #65064 ) ;
#115813=ORIENTED_EDGE ( 'NONE', *, *, #128049, .F. ) ;
#115814=CIRCLE ( 'NONE', #4987, 0.09999999999999982514 ) ;
#115815=EDGE_CURVE ( 'NONE', #62716, #83439, #11500, .T. ) ;
#115816=EDGE_CURVE ( 'NONE', #62036, #58504, #57373, .T. ) ;
#115817=DIRECTION ( 'NONE',  ( 0.000000000000000000, 1.000000000000000000, 0.000000000000000000 ) ) ;
#115818=VERTEX_POINT ( 'NONE', #92636 ) ;
#115819=EDGE_LOOP ( 'NONE', ( #102808, #50786 ) ) ;
#115820=FACE_OUTER_BOUND ( 'NONE', #98242, .T. ) ;
#115821=FACE_OUTER_BOUND ( 'NONE', #109333, .T. ) ;
#115822=DIRECTION ( 'NONE',  ( 0.000000000000000000, 0.000000000000000000, 1.000000000000000000 ) ) ;
#115823=DIRECTION ( 'NONE',  ( 0.000000000000000000, 0.000000000000000000, 1.000000000000000000 ) ) ;
#115824=CARTESIAN_POINT ( 'NONE',  ( 10.39999999999990976, 2.500000000000000000, -4.230127018922201998 ) ) ;
#115825=CIRCLE ( 'NONE', #80334, 0.1000000000000002554 ) ;
#115826=CARTESIAN_POINT ( 'NONE',  ( 4.149999999999939959, 2.500000000000000000, -2.165063509461101710 ) ) ;
#115827=CIRCLE ( 'NONE', #30168, 0.06509327318403745899 ) ;
#115828=CONICAL_SURFACE ( 'NONE', #7148, 0.1000000000000002554, 0.003490658503988666988 ) ;
#115829=DIRECTION ( 'NONE',  ( 0.000000000000000000, 0.000000000000000000, -1.000000000000000000 ) ) ;
#115830=ORIENTED_EDGE ( 'NONE', *, *, #13667, .T. ) ;
#115831=DIRECTION ( 'NONE',  ( 0.000000000000000000, 0.000000000000000000, 1.000000000000000000 ) ) ;
#115832=CIRCLE ( 'NONE', #36437, 0.06509327318403745899 ) ;
#115833=AXIS2_PLACEMENT_3D ( 'NONE', #117640, #71139, #83557 ) ;
#115834=FACE_OUTER_BOUND ( 'NONE', #122729, .T. ) ;
#115835=EDGE_LOOP ( 'NONE', ( #34215, #66693 ) ) ;
#115836=VERTEX_POINT ( 'NONE', #61906 ) ;
#115837=EDGE_LOOP ( 'NONE', ( #28086, #35267 ) ) ;
#115838=EDGE_LOOP ( 'NONE', ( #118218, #9975, #90747, #124286 ) ) ;
#115839=CARTESIAN_POINT ( 'NONE',  ( 1.849999999999951017, 2.500000000000000000, -6.248780366869526759 ) ) ;
#115840=DIRECTION ( 'NONE',  ( -4.274815082592931898E-19, -0.9999939076577903929, -0.003490651415223739937 ) ) ;
#115841=DIRECTION ( 'NONE',  ( 0.000000000000000000, 0.000000000000000000, -1.000000000000000000 ) ) ;
#115842=FACE_OUTER_BOUND ( 'NONE', #95464, .T. ) ;
#115843=VECTOR ( 'NONE', #96656, 1000.000000000000000 ) ;
#115844=CARTESIAN_POINT ( 'NONE',  ( 0.6499999999999566125, 2.500000000000000000, -6.741600689897077281 ) ) ;
#115845=ORIENTED_EDGE ( 'NONE', *, *, #41648, .F. ) ;
#115846=AXIS2_PLACEMENT_3D ( 'NONE', #43563, #80900, #91350 ) ;
#115847=AXIS2_PLACEMENT_3D ( 'NONE', #22754, #30635, #43048 ) ;
#115848=DIRECTION ( 'NONE',  ( -0.000000000000000000, 1.000000000000000000, -0.000000000000000000 ) ) ;
#115850=EDGE_CURVE ( 'NONE', #74354, #71030, #101820, .T. ) ;
#115851=EDGE_LOOP ( 'NONE', ( #48925, #8596 ) ) ;
#115852=CIRCLE ( 'NONE', #59451, 0.1000000000000002554 ) ;
#115853=AXIS2_PLACEMENT_3D ( 'NONE', #110343, #71066, #81532 ) ;
#115854=ORIENTED_EDGE ( 'NONE', *, *, #68302, .T. ) ;
#115855=AXIS2_PLACEMENT_3D ( 'NONE', #40003, #10510, #90359 ) ;
#115856=ORIENTED_EDGE ( 'NONE', *, *, #87035, .T. ) ;
#115857=CARTESIAN_POINT ( 'NONE',  ( 3.349999999999941913, 2.500000000000000000, 6.495190528383297135 ) ) ;
#115858=EDGE_CURVE ( 'NONE', #86174, #90407, #82175, .T. ) ;
#115859=DIRECTION ( 'NONE',  ( 0.000000000000000000, 0.000000000000000000, 1.000000000000000000 ) ) ;
#115860=CARTESIAN_POINT ( 'NONE',  ( 0.4499999999999552136, 2.500000000000000000, 6.395190528383296602 ) ) ;
#115861=AXIS2_PLACEMENT_3D ( 'NONE', #60033, #122167, #91396 ) ;
#115862=CIRCLE ( 'NONE', #38620, 0.1000000000000002554 ) ;
#115863=AXIS2_PLACEMENT_3D ( 'NONE', #26896, #115910, #64867 ) ;
#115864=AXIS2_PLACEMENT_3D ( 'NONE', #29400, #71235, #50317 ) ;
#115865=EDGE_CURVE ( 'NONE', #6379, #84904, #30203, .T. ) ;
#115866=ORIENTED_EDGE ( 'NONE', *, *, #71010, .T. ) ;
#115867=DIRECTION ( 'NONE',  ( 0.000000000000000000, 0.000000000000000000, 1.000000000000000000 ) ) ;
#115868=LINE ( 'NONE', #26205, #95618 ) ;
#115869=FACE_OUTER_BOUND ( 'NONE', #104635, .T. ) ;
#115870=CARTESIAN_POINT ( 'NONE',  ( -11.84999999999999609, 2.500000000000000000, 1.818653347947321475 ) ) ;
#115871=EDGE_CURVE ( 'NONE', #101758, #121980, #126619, .T. ) ;
#115872=DIRECTION ( 'NONE',  ( -0.000000000000000000, 1.000000000000000000, -0.000000000000000000 ) ) ;
#115873=EDGE_LOOP ( 'NONE', ( #422, #122323, #29165, #79588 ) ) ;
#115874=PLANE ( 'NONE',  #1877 ) ;
#115875=VERTEX_POINT ( 'NONE', #84752 ) ;
#115876=ORIENTED_EDGE ( 'NONE', *, *, #73089, .F. ) ;
#115877=VERTEX_POINT ( 'NONE', #125319 ) ;
#115878=EDGE_CURVE ( 'NONE', #9138, #107707, #120070, .T. ) ;
#115879=DIRECTION ( 'NONE',  ( -0.000000000000000000, -1.000000000000000000, -0.000000000000000000 ) ) ;
#115880=FACE_BOUND ( 'NONE', #67145, .T. ) ;
#115881=DIRECTION ( 'NONE',  ( -0.000000000000000000, 1.000000000000000000, -0.000000000000000000 ) ) ;
#115882=CIRCLE ( 'NONE', #957, 0.06509327318403745899 ) ;
#115883=FACE_OUTER_BOUND ( 'NONE', #56713, .T. ) ;
#115884=CARTESIAN_POINT ( 'NONE',  ( -8.950000000000008171, 2.500000000000000000, 1.918653347947321564 ) ) ;
#115885=ORIENTED_EDGE ( 'NONE', *, *, #39578, .T. ) ;
#115886=PLANE ( 'NONE',  #127524 ) ;
#115887=CARTESIAN_POINT ( 'NONE',  ( 11.84999999999990727, 2.500000000000000000, 6.248780366869520542 ) ) ;
#115888=CARTESIAN_POINT ( 'NONE',  ( 16.32066102237049066, 2.500000000000000000, 4.877377760480499980 ) ) ;
#115889=CARTESIAN_POINT ( 'NONE',  ( -14.99999999999994671, 12.50000000000000000, 0.06509327318403743123 ) ) ;
#115890=VERTEX_POINT ( 'NONE', #35031 ) ;
#115891=AXIS2_PLACEMENT_3D ( 'NONE', #123613, #33965, #105282 ) ;
#115892=CARTESIAN_POINT ( 'NONE',  ( -1.650000000000034772, 2.500000000000000000, 2.165063509461097713 ) ) ;
#115893=DIRECTION ( 'NONE',  ( -0.000000000000000000, -1.000000000000000000, -0.000000000000000000 ) ) ;
#115894=ORIENTED_EDGE ( 'NONE', *, *, #49119, .F. ) ;
#115895=CARTESIAN_POINT ( 'NONE',  ( 8.749999999999953815, 2.500000000000000000, -2.165063509461101710 ) ) ;
#115896=FACE_BOUND ( 'NONE', #57843, .T. ) ;
#115897=DIRECTION ( 'NONE',  ( 0.000000000000000000, 0.000000000000000000, 1.000000000000000000 ) ) ;
#115898=AXIS2_PLACEMENT_3D ( 'NONE', #1566, #21878, #29748 ) ;
#115899=EDGE_CURVE ( 'NONE', #124866, #79421, #14053, .T. ) ;
#115900=EDGE_LOOP ( 'NONE', ( #52924, #26252, #123393, #112561 ) ) ;
#115901=CARTESIAN_POINT ( 'NONE',  ( 4.799999999999934097, 2.500000000000000000, 4.676537180435972552 ) ) ;
#115902=CARTESIAN_POINT ( 'NONE',  ( 12.04999999999990834, 12.50000000000000000, 6.495190528383297135 ) ) ;
#115903=AXIS2_PLACEMENT_3D ( 'NONE', #119142, #39326, #79230 ) ;
#115904=ORIENTED_EDGE ( 'NONE', *, *, #57587, .T. ) ;
#115905=ORIENTED_EDGE ( 'NONE', *, *, #49612, .T. ) ;
#115906=EDGE_CURVE ( 'NONE', #17226, #85840, #113813, .T. ) ;
#115908=EDGE_CURVE ( 'NONE', #48001, #26422, #6797, .T. ) ;
#115909=ORIENTED_EDGE ( 'NONE', *, *, #112829, .F. ) ;
#115910=DIRECTION ( 'NONE',  ( -0.000000000000000000, 1.000000000000000000, -0.000000000000000000 ) ) ;
#115911=DIRECTION ( 'NONE',  ( -0.000000000000000000, -1.000000000000000000, -0.000000000000000000 ) ) ;
#115912=AXIS2_PLACEMENT_3D ( 'NONE', #128314, #129613, #39931 ) ;
#115913=CONICAL_SURFACE ( 'NONE', #92951, 0.1000000000000002554, 0.003490658503988666988 ) ;
#115914=DIRECTION ( 'NONE',  ( -0.000000000000000000, 1.000000000000000000, -0.000000000000000000 ) ) ;
#115915=DIRECTION ( 'NONE',  ( 0.000000000000000000, 0.000000000000000000, 1.000000000000000000 ) ) ;
#115916=ADVANCED_FACE ( 'NONE', ( #86680 ), #117998, .T. ) ;
#115917=EDGE_CURVE ( 'NONE', #50837, #30524, #56561, .T. ) ;
#115918=CONICAL_SURFACE ( 'NONE', #59525, 0.1000000000000002554, 0.003490658503988666988 ) ;
#115919=CARTESIAN_POINT ( 'NONE',  ( 8.949999999999915801, 2.500000000000000000, -1.818653347947326138 ) ) ;
#115920=EDGE_CURVE ( 'NONE', #73436, #104132, #78319, .T. ) ;
#115921=AXIS2_PLACEMENT_3D ( 'NONE', #76949, #68401, #129294 ) ;
#115922=ORIENTED_EDGE ( 'NONE', *, *, #96650, .F. ) ;
#115923=DIRECTION ( 'NONE',  ( 0.000000000000000000, 0.000000000000000000, 1.000000000000000000 ) ) ;
#115924=ADVANCED_FACE ( 'NONE', ( #65745 ), #11492, .T. ) ;
#115925=PLANE ( 'NONE',  #9993 ) ;
#115926=FACE_OUTER_BOUND ( 'NONE', #101314, .T. ) ;
#115927=PLANE ( 'NONE',  #109674 ) ;
#115929=EDGE_LOOP ( 'NONE', ( #88818, #18552 ) ) ;
#115930=FACE_OUTER_BOUND ( 'NONE', #31750, .T. ) ;
#115932=CARTESIAN_POINT ( 'NONE',  ( 0.3999999999999628852, 2.500000000000000000, -0.6928203230275520319 ) ) ;
#115933=CARTESIAN_POINT ( 'NONE',  ( 3.549999999999942979, 12.50000000000000000, 1.818653347947321475 ) ) ;
#115934=EDGE_CURVE ( 'NONE', #89926, #83615, #38614, .T. ) ;
#115935=ORIENTED_EDGE ( 'NONE', *, *, #57203, .F. ) ;
#115936=CARTESIAN_POINT ( 'NONE',  ( 7.299999999999927880, 2.500000000000000000, -4.576537180435977348 ) ) ;
#115937=CARTESIAN_POINT ( 'NONE',  ( 10.19999999999991402, 2.500000000000000000, 0.4464101615137735513 ) ) ;
#115938=DIRECTION ( 'NONE',  ( 0.000000000000000000, 0.000000000000000000, -1.000000000000000000 ) ) ;
#115939=CARTESIAN_POINT ( 'NONE',  ( -10.84999999999999964, 12.50000000000000000, 5.867463478539781896 ) ) ;
#115940=ORIENTED_EDGE ( 'NONE', *, *, #91041, .F. ) ;
#115941=AXIS2_PLACEMENT_3D ( 'NONE', #39076, #391, #8286 ) ;
#115942=DIRECTION ( 'NONE',  ( 0.000000000000000000, 0.000000000000000000, 1.000000000000000000 ) ) ;
#115943=DIRECTION ( 'NONE',  ( 0.000000000000000000, 0.000000000000000000, 1.000000000000000000 ) ) ;
#115944=CONICAL_SURFACE ( 'NONE', #105489, 0.1000000000000002554, 0.003490658503988666988 ) ;
#115945=CIRCLE ( 'NONE', #122214, 0.06509327318403741736 ) ;
#115946=CARTESIAN_POINT ( 'NONE',  ( 11.44999999999991047, 2.500000000000000000, 6.048780366869520364 ) ) ;
#115948=CARTESIAN_POINT ( 'NONE',  ( -0.8500000000000386136, 2.500000000000000000, 2.957883832488649389 ) ) ;
#115949=AXIS2_PLACEMENT_3D ( 'NONE', #10366, #119667, #48358 ) ;
#115950=EDGE_LOOP ( 'NONE', ( #83967, #56717 ) ) ;
#115951=CONICAL_SURFACE ( 'NONE', #34497, 0.1000000000000002554, 0.003490658503988666988 ) ;
#115952=ORIENTED_EDGE ( 'NONE', *, *, #124515, .T. ) ;
#115953=VECTOR ( 'NONE', #124024, 1000.000000000000000 ) ;
#115954=CARTESIAN_POINT ( 'NONE',  ( -9.200000000000009948, 2.500000000000000000, -4.430127018922197735 ) ) ;
#115955=VERTEX_POINT ( 'NONE', #105685 ) ;
#115956=CARTESIAN_POINT ( 'NONE',  ( -9.800000000000004263, 2.500000000000000000, -0.3464101615137783474 ) ) ;
#115957=CIRCLE ( 'NONE', #19819, 0.06509327318403743123 ) ;
#115958=VERTEX_POINT ( 'NONE', #63829 ) ;
#115959=VERTEX_POINT ( 'NONE', #75563 ) ;
#115960=ORIENTED_EDGE ( 'NONE', *, *, #71614, .F. ) ;
#115961=DIRECTION ( 'NONE',  ( 0.000000000000000000, 0.000000000000000000, 1.000000000000000000 ) ) ;
#115962=CARTESIAN_POINT ( 'NONE',  ( -12.29999999999999361, 12.50000000000000000, 3.983716857408420076 ) ) ;
#115963=DIRECTION ( 'NONE',  ( -4.274815082592931898E-19, -0.9999939076577903929, -0.003490651415223739937 ) ) ;
#115964=DIRECTION ( 'NONE',  ( 0.000000000000000000, -0.9999939076577903929, 0.003490651415223739937 ) ) ;
#115965=CARTESIAN_POINT ( 'NONE',  ( 6.249999999999967137, 2.500000000000000000, 6.495190528383297135 ) ) ;
#115966=CIRCLE ( 'NONE', #5143, 0.1000000000000002554 ) ;
#115967=DIRECTION ( 'NONE',  ( 0.000000000000000000, 0.000000000000000000, 1.000000000000000000 ) ) ;
#115968=EDGE_LOOP ( 'NONE', ( #101173, #61800, #88242, #111748 ) ) ;
#115969=FACE_OUTER_BOUND ( 'NONE', #31752, .T. ) ;
#115970=EDGE_LOOP ( 'NONE', ( #99188, #12535, #24038, #124744 ) ) ;
#115971=ORIENTED_EDGE ( 'NONE', *, *, #78087, .T. ) ;
#115972=ORIENTED_EDGE ( 'NONE', *, *, #5263, .T. ) ;
#115973=EDGE_CURVE ( 'NONE', #97073, #28400, #105017, .T. ) ;
#115974=ORIENTED_EDGE ( 'NONE', *, *, #115511, .T. ) ;
#115975=FACE_OUTER_BOUND ( 'NONE', #65566, .T. ) ;
#115977=VERTEX_POINT ( 'NONE', #115471 ) ;
#115978=VECTOR ( 'NONE', #108187, 1000.000000000000000 ) ;
#115979=EDGE_CURVE ( 'NONE', #122022, #74917, #122321, .T. ) ;
#115981=CARTESIAN_POINT ( 'NONE',  ( -5.400000000000023448, 2.500000000000000000, -4.430127018922202176 ) ) ;
#115982=CARTESIAN_POINT ( 'NONE',  ( -11.89999999999999680, 12.50000000000000000, -4.048810130592460865 ) ) ;
#115983=LINE ( 'NONE', #77353, #43009 ) ;
#115984=CARTESIAN_POINT ( 'NONE',  ( 12.94999999999990337, 2.500000000000000000, 2.165063509461097713 ) ) ;
#115985=ORIENTED_EDGE ( 'NONE', *, *, #16984, .T. ) ;
#115986=CARTESIAN_POINT ( 'NONE',  ( 8.299999999999922551, 2.500000000000000000, -4.330127018922201643 ) ) ;
#115987=CIRCLE ( 'NONE', #120202, 0.09999999999999982514 ) ;
#115988=CONICAL_SURFACE ( 'NONE', #47043, 0.1000000000000002554, 0.003490658503988666988 ) ;
#115989=ORIENTED_EDGE ( 'NONE', *, *, #125628, .T. ) ;
#115990=DIRECTION ( 'NONE',  ( -4.274815082592931898E-19, -0.9999939076577903929, -0.003490651415223739937 ) ) ;
#115991=ORIENTED_EDGE ( 'NONE', *, *, #9375, .F. ) ;
#115992=DIRECTION ( 'NONE',  ( -0.000000000000000000, 1.000000000000000000, -0.000000000000000000 ) ) ;
#115993=ORIENTED_EDGE ( 'NONE', *, *, #124639, .F. ) ;
#115994=VERTEX_POINT ( 'NONE', #25832 ) ;
#115995=DIRECTION ( 'NONE',  ( 0.000000000000000000, 0.000000000000000000, 1.000000000000000000 ) ) ;
#115996=CARTESIAN_POINT ( 'NONE',  ( 4.999999999999973355, 2.500000000000000000, -4.430127018922202176 ) ) ;
#115997=DIRECTION ( 'NONE',  ( 0.000000000000000000, 0.000000000000000000, 1.000000000000000000 ) ) ;
#115998=DIRECTION ( 'NONE',  ( 0.000000000000000000, 0.000000000000000000, 1.000000000000000000 ) ) ;
#115999=CONICAL_SURFACE ( 'NONE', #103483, 0.1000000000000002554, 0.003490658503988666988 ) ;
#116000=DIRECTION ( 'NONE',  ( -0.000000000000000000, -1.000000000000000000, -0.000000000000000000 ) ) ;
#116001=EDGE_LOOP ( 'NONE', ( #96217, #718, #68025, #123484 ) ) ;
#116002=DIRECTION ( 'NONE',  ( 0.000000000000000000, 0.000000000000000000, 1.000000000000000000 ) ) ;
#116003=CARTESIAN_POINT ( 'NONE',  ( 6.699999999999930012, 2.500000000000000000, -4.330127018922201643 ) ) ;
#116004=CARTESIAN_POINT ( 'NONE',  ( -6.250000000000021316, 2.500000000000000000, -1.372243186433550033 ) ) ;
#116005=DIRECTION ( 'NONE',  ( 0.000000000000000000, 1.000000000000000000, 0.000000000000000000 ) ) ;
#116006=DIRECTION ( 'NONE',  ( 0.000000000000000000, 1.000000000000000000, 0.000000000000000000 ) ) ;
#116008=ORIENTED_EDGE ( 'NONE', *, *, #5841, .F. ) ;
#116009=CONICAL_SURFACE ( 'NONE', #59609, 0.09999999999999982514, 0.003490658503988666988 ) ;
#116010=AXIS2_PLACEMENT_3D ( 'NONE', #99198, #38348, #58634 ) ;
#116011=ORIENTED_EDGE ( 'NONE', *, *, #66694, .F. ) ;
#116012=PLANE ( 'NONE',  #90294 ) ;
#116013=VERTEX_POINT ( 'NONE', #103752 ) ;
#116014=CARTESIAN_POINT ( 'NONE',  ( 10.39999999999991331, 2.500000000000000000, -2.385244779468109755E-15 ) ) ;
#116015=FACE_OUTER_BOUND ( 'NONE', #8704, .T. ) ;
#116016=ADVANCED_FACE ( 'NONE', ( #44840 ), #65863, .T. ) ;
#116017=ADVANCED_FACE ( 'NONE', ( #85393 ), #86709, .T. ) ;
#116018=VERTEX_POINT ( 'NONE', #116134 ) ;
#116020=DIRECTION ( 'NONE',  ( 0.000000000000000000, 0.000000000000000000, 1.000000000000000000 ) ) ;
#116021=DIRECTION ( 'NONE',  ( 0.000000000000000000, 0.000000000000000000, 1.000000000000000000 ) ) ;
#116022=DIRECTION ( 'NONE',  ( 0.000000000000000000, 0.000000000000000000, 1.000000000000000000 ) ) ;
#116023=EDGE_CURVE ( 'NONE', #22314, #107468, #6171, .T. ) ;
#116024=CIRCLE ( 'NONE', #124438, 0.06509327318403745899 ) ;
#116025=FACE_OUTER_BOUND ( 'NONE', #44148, .T. ) ;
#116026=ORIENTED_EDGE ( 'NONE', *, *, #26445, .T. ) ;
#116027=AXIS2_PLACEMENT_3D ( 'NONE', #49467, #42213, #79553 ) ;
#116028=DIRECTION ( 'NONE',  ( -0.000000000000000000, 1.000000000000000000, -0.000000000000000000 ) ) ;
#116029=LINE ( 'NONE', #26376, #106170 ) ;
#116030=ADVANCED_FACE ( 'NONE', ( #66393 ), #49170, .T. ) ;
#116031=AXIS2_PLACEMENT_3D ( 'NONE', #88639, #78187, #128594 ) ;
#116032=ORIENTED_EDGE ( 'NONE', *, *, #6084, .T. ) ;
#116033=AXIS2_PLACEMENT_3D ( 'NONE', #115273, #26932, #74748 ) ;
#116034=EDGE_CURVE ( 'NONE', #71376, #76654, #15675, .T. ) ;
#116035=DIRECTION ( 'NONE',  ( 0.000000000000000000, 1.000000000000000000, 0.000000000000000000 ) ) ;
#116036=CARTESIAN_POINT ( 'NONE',  ( -15.39999999999998082, 12.50000000000000000, 0.6928203230275518099 ) ) ;
#116037=DIRECTION ( 'NONE',  ( -0.000000000000000000, -1.000000000000000000, -0.000000000000000000 ) ) ;
#116038=CIRCLE ( 'NONE', #36648, 0.06509327318403745899 ) ;
#116039=EDGE_LOOP ( 'NONE', ( #80690, #113045 ) ) ;
#116040=CIRCLE ( 'NONE', #1112, 0.1000000000000002554 ) ;
#116041=FACE_OUTER_BOUND ( 'NONE', #6063, .T. ) ;
#116042=AXIS2_PLACEMENT_3D ( 'NONE', #104584, #44372, #72567 ) ;
#116043=VERTEX_POINT ( 'NONE', #109552 ) ;
#116044=DIRECTION ( 'NONE',  ( 0.000000000000000000, -0.9999939076577903929, 0.003490651415223739937 ) ) ;
#116045=DIRECTION ( 'NONE',  ( -0.000000000000000000, -1.000000000000000000, -0.000000000000000000 ) ) ;
#116046=CARTESIAN_POINT ( 'NONE',  ( 4.399999999999939071, 2.500000000000000000, 0.3464101615137736845 ) ) ;
#116047=ORIENTED_EDGE ( 'NONE', *, *, #22113, .T. ) ;
#116048=AXIS2_PLACEMENT_3D ( 'NONE', #50171, #61925, #120191 ) ;
#116049=AXIS2_PLACEMENT_3D ( 'NONE', #85968, #76819, #115416 ) ;
#116050=DIRECTION ( 'NONE',  ( 0.000000000000000000, 0.000000000000000000, -1.000000000000000000 ) ) ;
#116051=CARTESIAN_POINT ( 'NONE',  ( 13.29999999999990301, 12.50000000000000000, -4.330127018922201643 ) ) ;
#116052=AXIS2_PLACEMENT_3D ( 'NONE', #4737, #125187, #74801 ) ;
#116053=VERTEX_POINT ( 'NONE', #19889 ) ;
#116054=ORIENTED_EDGE ( 'NONE', *, *, #117221, .F. ) ;
#116055=CARTESIAN_POINT ( 'NONE',  ( 4.599999999999935696, 2.500000000000000000, 5.022947341949748790 ) ) ;
#116056=EDGE_LOOP ( 'NONE', ( #39866, #37562 ) ) ;
#116058=CARTESIAN_POINT ( 'NONE',  ( -11.64999999999999680, 2.500000000000000000, -6.495190528383298911 ) ) ;
#116059=ORIENTED_EDGE ( 'NONE', *, *, #43261, .F. ) ;
#116060=PLANE ( 'NONE',  #48866 ) ;
#116061=FACE_OUTER_BOUND ( 'NONE', #89622, .T. ) ;
#116062=AXIS2_PLACEMENT_3D ( 'NONE', #119298, #109491, #19828 ) ;
#116063=ORIENTED_EDGE ( 'NONE', *, *, #123702, .F. ) ;
#116064=EDGE_CURVE ( 'NONE', #54722, #29933, #27752, .T. ) ;
#116065=DIRECTION ( 'NONE',  ( 0.000000000000000000, 0.000000000000000000, 1.000000000000000000 ) ) ;
#116067=EDGE_CURVE ( 'NONE', #110791, #63955, #82606, .T. ) ;
#116068=DIRECTION ( 'NONE',  ( 0.000000000000000000, 0.000000000000000000, -1.000000000000000000 ) ) ;
#116069=DIRECTION ( 'NONE',  ( 0.000000000000000000, 1.000000000000000000, 0.000000000000000000 ) ) ;
#116070=EDGE_CURVE ( 'NONE', #36428, #116703, #97150, .T. ) ;
#116071=CARTESIAN_POINT ( 'NONE',  ( 11.24999999999994493, 12.50000000000000000, 6.430097255199259010 ) ) ;
#116072=CONICAL_SURFACE ( 'NONE', #59677, 0.1000000000000000472, 0.003490658503988666988 ) ;
#116073=CARTESIAN_POINT ( 'NONE',  ( 7.499999999999925393, 12.50000000000000000, -0.6928203230275541413 ) ) ;
#116074=EDGE_CURVE ( 'NONE', #4955, #99447, #10061, .T. ) ;
#116075=EDGE_CURVE ( 'NONE', #54276, #7138, #109703, .T. ) ;
#116076=AXIS2_PLACEMENT_3D ( 'NONE', #29788, #300, #118807 ) ;
#116077=ORIENTED_EDGE ( 'NONE', *, *, #62030, .F. ) ;
#116078=EDGE_LOOP ( 'NONE', ( #119807, #79443, #8060, #92655 ) ) ;
#116079=EDGE_CURVE ( 'NONE', #105882, #126334, #34498, .T. ) ;
#116080=ORIENTED_EDGE ( 'NONE', *, *, #23827, .T. ) ;
#116081=ORIENTED_EDGE ( 'NONE', *, *, #58817, .T. ) ;
#116082=CARTESIAN_POINT ( 'NONE',  ( 87.50000000000001421, 3.975350567648425759, 6.360562287258741065 ) ) ;
#116084=CARTESIAN_POINT ( 'NONE',  ( 12.94999999999989981, 2.500000000000000000, -2.165063509461101710 ) ) ;
#116085=VERTEX_POINT ( 'NONE', #118718 ) ;
#116086=FACE_BOUND ( 'NONE', #114632, .T. ) ;
#116087=DIRECTION ( 'NONE',  ( 0.000000000000000000, 1.000000000000000000, 0.000000000000000000 ) ) ;
#116088=DIRECTION ( 'NONE',  ( 0.000000000000000000, -0.9999939076577903929, 0.003490651415223739937 ) ) ;
#116089=EDGE_CURVE ( 'NONE', #55907, #64926, #120161, .T. ) ;
#116090=DIRECTION ( 'NONE',  ( -0.000000000000000000, -1.000000000000000000, -0.000000000000000000 ) ) ;
#116091=EDGE_CURVE ( 'NONE', #96832, #46254, #61680, .T. ) ;
#116092=LINE ( 'NONE', #34983, #26227 ) ;
#116093=CIRCLE ( 'NONE', #59692, 0.09999999999999982514 ) ;
#116094=CARTESIAN_POINT ( 'NONE',  ( 17.49862860983166257, -2.500000000000000000, -4.081131818001380474 ) ) ;
#116095=DIRECTION ( 'NONE',  ( 0.000000000000000000, 1.000000000000000000, 0.000000000000000000 ) ) ;
#116096=DIRECTION ( 'NONE',  ( -0.000000000000000000, -1.000000000000000000, -0.000000000000000000 ) ) ;
#116097=CARTESIAN_POINT ( 'NONE',  ( -10.84999999999999964, 12.50000000000000000, 5.802370205355744659 ) ) ;
#116098=CARTESIAN_POINT ( 'NONE',  ( 4.599999999999938360, 2.500000000000000000, -0.6928203230275541413 ) ) ;
#116099=DIRECTION ( 'NONE',  ( 0.000000000000000000, 0.000000000000000000, 1.000000000000000000 ) ) ;
#116100=ORIENTED_EDGE ( 'NONE', *, *, #115710, .T. ) ;
#116101=VERTEX_POINT ( 'NONE', #79456 ) ;
#116102=CIRCLE ( 'NONE', #111906, 0.06509327318403745899 ) ;
#116103=ORIENTED_EDGE ( 'NONE', *, *, #113396, .F. ) ;
#116104=EDGE_LOOP ( 'NONE', ( #55111, #86880 ) ) ;
#116105=DIRECTION ( 'NONE',  ( 0.000000000000000000, 0.000000000000000000, -1.000000000000000000 ) ) ;
#116106=ORIENTED_EDGE ( 'NONE', *, *, #95109, .T. ) ;
#116107=CARTESIAN_POINT ( 'NONE',  ( 5.449999999999936229, 2.500000000000000000, 6.595190528383296780 ) ) ;
#116108=ORIENTED_EDGE ( 'NONE', *, *, #45132, .F. ) ;
#116109=ORIENTED_EDGE ( 'NONE', *, *, #113546, .F. ) ;
#116110=DIRECTION ( 'NONE',  ( 0.000000000000000000, 1.000000000000000000, 0.000000000000000000 ) ) ;
#116112=DIRECTION ( 'NONE',  ( 0.000000000000000000, -0.9999939076577903929, 0.003490651415223739937 ) ) ;
#116113=LINE ( 'NONE', #118045, #83477 ) ;
#116115=CARTESIAN_POINT ( 'NONE',  ( -4.600000000000028066, 12.50000000000000000, -3.572213422710612374 ) ) ;
#116116=ORIENTED_EDGE ( 'NONE', *, *, #93787, .F. ) ;
#116117=EDGE_LOOP ( 'NONE', ( #91118, #125305 ) ) ;
#116118=VECTOR ( 'NONE', #40124, 1000.000000000000000 ) ;
#116119=ORIENTED_EDGE ( 'NONE', *, *, #30396, .F. ) ;
#116120=ORIENTED_EDGE ( 'NONE', *, *, #17796, .F. ) ;
#116121=AXIS2_PLACEMENT_3D ( 'NONE', #81412, #112152, #121318 ) ;
#116122=CARTESIAN_POINT ( 'NONE',  ( 5.599999999999934808, 12.50000000000000000, -4.611443907251940644 ) ) ;
#116123=ORIENTED_EDGE ( 'NONE', *, *, #104545, .F. ) ;
#116124=ORIENTED_EDGE ( 'NONE', *, *, #105266, .F. ) ;
#116125=LINE ( 'NONE', #8106, #86079 ) ;
#116126=AXIS2_PLACEMENT_3D ( 'NONE', #96327, #127733, #48539 ) ;
#116127=EDGE_CURVE ( 'NONE', #53696, #53628, #57220, .T. ) ;
#116128=CARTESIAN_POINT ( 'NONE',  ( -4.800000000000024691, 2.500000000000000000, 0.3464101615137735735 ) ) ;
#116129=DIRECTION ( 'NONE',  ( -0.000000000000000000, 1.000000000000000000, -0.000000000000000000 ) ) ;
#116130=CARTESIAN_POINT ( 'NONE',  ( -5.000000000000022204, 2.500000000000000000, -0.6928203230275541413 ) ) ;
#116132=DIRECTION ( 'NONE',  ( 0.000000000000000000, 1.000000000000000000, 0.000000000000000000 ) ) ;
#116133=EDGE_LOOP ( 'NONE', ( #4502, #36592 ) ) ;
#116134=CARTESIAN_POINT ( 'NONE',  ( -12.29999999999999716, 2.500000000000000000, -4.083716857408424161 ) ) ;
#116135=AXIS2_PLACEMENT_3D ( 'NONE', #8131, #87965, #37617 ) ;
#116136=CIRCLE ( 'NONE', #9543, 0.09999999999999982514 ) ;
#116137=ORIENTED_EDGE ( 'NONE', *, *, #119170, .F. ) ;
#116138=FACE_OUTER_BOUND ( 'NONE', #29433, .T. ) ;
#116139=ORIENTED_EDGE ( 'NONE', *, *, #86183, .F. ) ;
#116141=CYLINDRICAL_SURFACE ( 'NONE', #80453, 1.000000000000000888 ) ;
#116142=CIRCLE ( 'NONE', #78520, 0.1000000000000000472 ) ;
#116143=ORIENTED_EDGE ( 'NONE', *, *, #39093, .T. ) ;
#116144=PLANE ( 'NONE',  #88537 ) ;
#116146=ORIENTED_EDGE ( 'NONE', *, *, #106619, .T. ) ;
#116147=DIRECTION ( 'NONE',  ( 0.000000000000000000, 1.000000000000000000, 0.000000000000000000 ) ) ;
#116148=EDGE_LOOP ( 'NONE', ( #110825, #111422 ) ) ;
#116149=ORIENTED_EDGE ( 'NONE', *, *, #22743, .T. ) ;
#116150=CARTESIAN_POINT ( 'NONE',  ( 8.349999999999923261, 2.500000000000000000, -5.902370205355750521 ) ) ;
#116151=CARTESIAN_POINT ( 'NONE',  ( -3.950000000000026379, 12.50000000000000000, -1.883746621131363597 ) ) ;
#116153=AXIS2_PLACEMENT_3D ( 'NONE', #108034, #118497, #1306 ) ;
#116154=CARTESIAN_POINT ( 'NONE',  ( -1.450000000000035927, 2.500000000000000000, -1.818653347947326138 ) ) ;
#116155=DIRECTION ( 'NONE',  ( 0.000000000000000000, 0.000000000000000000, 1.000000000000000000 ) ) ;
#116156=DIRECTION ( 'NONE',  ( 0.000000000000000000, 0.000000000000000000, -1.000000000000000000 ) ) ;
#116157=VECTOR ( 'NONE', #19003, 1000.000000000000000 ) ;
#116158=CONICAL_SURFACE ( 'NONE', #63948, 0.1000000000000000472, 0.003490658503988666988 ) ;
#116159=ORIENTED_EDGE ( 'NONE', *, *, #14034, .F. ) ;
#116160=AXIS2_PLACEMENT_3D ( 'NONE', #102400, #123320, #71643 ) ;
#116161=DIRECTION ( 'NONE',  ( 0.000000000000000000, 0.000000000000000000, 1.000000000000000000 ) ) ;
#116162=EDGE_CURVE ( 'NONE', #104463, #20844, #72137, .T. ) ;
#116163=AXIS2_PLACEMENT_3D ( 'NONE', #24305, #122510, #14460 ) ;
#116164=ORIENTED_EDGE ( 'NONE', *, *, #5105, .F. ) ;
#116165=EDGE_CURVE ( 'NONE', #31641, #32791, #99241, .T. ) ;
#116166=CARTESIAN_POINT ( 'NONE',  ( 9.349999999999916156, 12.50000000000000000, 6.213873640053558134 ) ) ;
#116167=DIRECTION ( 'NONE',  ( 0.000000000000000000, 1.000000000000000000, 0.000000000000000000 ) ) ;
#116168=DIRECTION ( 'NONE',  ( 0.000000000000000000, 0.000000000000000000, 1.000000000000000000 ) ) ;
#116169=ADVANCED_FACE ( 'NONE', ( #88617 ), #107615, .T. ) ;
#116170=ORIENTED_EDGE ( 'NONE', *, *, #40699, .T. ) ;
#116171=VECTOR ( 'NONE', #103987, 1000.000000000000000 ) ;
#116172=AXIS2_PLACEMENT_3D ( 'NONE', #67116, #107062, #47524 ) ;
#116173=CARTESIAN_POINT ( 'NONE',  ( -4.150000000000027889, 2.500000000000000000, -7.288010851410854585 ) ) ;
#116174=CARTESIAN_POINT ( 'NONE',  ( -9.150000000000009237, 12.50000000000000000, -6.560283801567334372 ) ) ;
#116175=EDGE_CURVE ( 'NONE', #62091, #94991, #29701, .T. ) ;
#116176=EDGE_CURVE ( 'NONE', #60290, #38624, #111850, .T. ) ;
#116177=ADVANCED_FACE ( 'NONE', ( #98416 ), #76256, .T. ) ;
#116178=EDGE_CURVE ( 'NONE', #49457, #54499, #103440, .T. ) ;
#116179=ORIENTED_EDGE ( 'NONE', *, *, #61725, .F. ) ;
#116180=DIRECTION ( 'NONE',  ( -0.000000000000000000, -1.000000000000000000, -0.000000000000000000 ) ) ;
#116181=CIRCLE ( 'NONE', #99486, 0.1000000000000002554 ) ;
#116182=CIRCLE ( 'NONE', #126665, 0.09999999999999982514 ) ;
#116183=ORIENTED_EDGE ( 'NONE', *, *, #28434, .T. ) ;
#116184=B_SPLINE_CURVE_WITH_KNOTS ( 'NONE', 3,
 ( #6101, #76801, #105618, #125877, #76157, #6728, #94485, #84678 ),
 .UNSPECIFIED., .F., .F.,
 ( 4, 2, 2, 4 ),
 ( -1.045402497998345297E-05, 0.001241257413632291563, 0.001867113132938430118, 0.002492968852244568673 ),
 .UNSPECIFIED. ) ;
#116185=ORIENTED_EDGE ( 'NONE', *, *, #57850, .T. ) ;
#116187=EDGE_CURVE ( 'NONE', #98794, #109646, #88856, .T. ) ;
#116189=DIRECTION ( 'NONE',  ( 0.000000000000000000, 1.000000000000000000, 0.000000000000000000 ) ) ;
#116190=CARTESIAN_POINT ( 'NONE',  ( 13.29999999999989946, 12.50000000000000000, -2.385244779468109755E-15 ) ) ;
#116191=CARTESIAN_POINT ( 'NONE',  ( 10.64999999999990976, 2.500000000000000000, -6.048780366869526581 ) ) ;
#116192=ORIENTED_EDGE ( 'NONE', *, *, #94940, .T. ) ;
#116193=FACE_BOUND ( 'NONE', #34665, .T. ) ;
#116194=DIRECTION ( 'NONE',  ( -0.000000000000000000, 1.000000000000000000, -0.000000000000000000 ) ) ;
#116195=VERTEX_POINT ( 'NONE', #120015 ) ;
#116196=LINE ( 'NONE', #44235, #67376 ) ;
#116197=CARTESIAN_POINT ( 'NONE',  ( -10.20000000000000462, 2.500000000000000000, 0.4464101615137735513 ) ) ;
#116198=ORIENTED_EDGE ( 'NONE', *, *, #51175, .T. ) ;
#116199=CONICAL_SURFACE ( 'NONE', #112118, 0.09999999999999982514, 0.003490658503988666988 ) ;
#116200=VERTEX_POINT ( 'NONE', #22481 ) ;
#116201=CONICAL_SURFACE ( 'NONE', #105756, 0.1000000000000002554, 0.003490658503988666988 ) ;
#116202=EDGE_LOOP ( 'NONE', ( #63800, #106341, #113522, #105478 ) ) ;
#116203=DIRECTION ( 'NONE',  ( 0.000000000000000000, 0.000000000000000000, 1.000000000000000000 ) ) ;
#116204=CARTESIAN_POINT ( 'NONE',  ( -9.999999999999971578, 12.50000000000000000, -4.395220292106235327 ) ) ;
#116205=DIRECTION ( 'NONE',  ( 0.000000000000000000, 0.000000000000000000, 1.000000000000000000 ) ) ;
#116206=EDGE_CURVE ( 'NONE', #105571, #28898, #126425, .T. ) ;
#116207=FACE_BOUND ( 'NONE', #51364, .T. ) ;
#116208=ORIENTED_EDGE ( 'NONE', *, *, #52512, .T. ) ;
#116210=CARTESIAN_POINT ( 'NONE',  ( -8.550000000000011369, 2.500000000000000000, -2.511473670974877948 ) ) ;
#116211=DIRECTION ( 'NONE',  ( 0.000000000000000000, 0.000000000000000000, 1.000000000000000000 ) ) ;
#116212=CIRCLE ( 'NONE', #11957, 0.06509327318403745899 ) ;
#116213=CARTESIAN_POINT ( 'NONE',  ( 6.449999999999928235, 2.500000000000000000, 2.511473670974873507 ) ) ;
#116214=PLANE ( 'NONE',  #54935 ) ;
#116215=EDGE_CURVE ( 'NONE', #1788, #26160, #55409, .T. ) ;
#116216=PLANE ( 'NONE',  #15447 ) ;
#116217=ADVANCED_FACE ( 'NONE', ( #21157 ), #80464, .T. ) ;
#116218=FACE_OUTER_BOUND ( 'NONE', #96111, .T. ) ;
#116219=DIRECTION ( 'NONE',  ( 0.000000000000000000, 0.000000000000000000, -1.000000000000000000 ) ) ;
#116220=EDGE_CURVE ( 'NONE', #58440, #27222, #12623, .T. ) ;
#116221=AXIS2_PLACEMENT_3D ( 'NONE', #82702, #104880, #73493 ) ;
#116222=FACE_OUTER_BOUND ( 'NONE', #102064, .T. ) ;
#116223=EDGE_CURVE ( 'NONE', #112402, #122474, #7271, .T. ) ;
#116224=VECTOR ( 'NONE', #76045, 1000.000000000000000 ) ;
#116225=ORIENTED_EDGE ( 'NONE', *, *, #3858, .T. ) ;
#116226=ORIENTED_EDGE ( 'NONE', *, *, #27193, .T. ) ;
#116227=ORIENTED_EDGE ( 'NONE', *, *, #57930, .F. ) ;
#116228=VERTEX_POINT ( 'NONE', #110197 ) ;
#116229=ORIENTED_EDGE ( 'NONE', *, *, #11331, .T. ) ;
#116230=CARTESIAN_POINT ( 'NONE',  ( -8.300000000000009592, 2.500000000000000000, 4.330127018922196314 ) ) ;
#116231=LINE ( 'NONE', #114305, #40364 ) ;
#116232=ORIENTED_EDGE ( 'NONE', *, *, #31583, .T. ) ;
#116233=ADVANCED_FACE ( 'NONE', ( #62393 ), #28224, .T. ) ;
#116234=FACE_BOUND ( 'NONE', #81820, .T. ) ;
#116235=CARTESIAN_POINT ( 'NONE',  ( -1.900000000000034106, 2.500000000000000000, -3.983716857408426293 ) ) ;
#116236=EDGE_CURVE ( 'NONE', #14247, #105063, #44950, .T. ) ;
#116237=EDGE_CURVE ( 'NONE', #67840, #122473, #91195, .T. ) ;
#116238=EDGE_CURVE ( 'NONE', #22180, #31609, #7363, .T. ) ;
#116239=CARTESIAN_POINT ( 'NONE',  ( 8.299999999999922551, 2.500000000000000000, 4.330127018922196314 ) ) ;
#116240=FACE_OUTER_BOUND ( 'NONE', #93767, .T. ) ;
#116241=DIRECTION ( 'NONE',  ( 0.000000000000000000, 0.000000000000000000, 1.000000000000000000 ) ) ;
#116242=CIRCLE ( 'NONE', #49381, 0.1000000000000000472 ) ;
#116243=ORIENTED_EDGE ( 'NONE', *, *, #72222, .T. ) ;
#116244=CARTESIAN_POINT ( 'NONE',  ( -6.450000000000014388, 2.500000000000000000, 6.248780366869521430 ) ) ;
#116245=EDGE_CURVE ( 'NONE', #55738, #61538, #80744, .T. ) ;
#116246=EDGE_LOOP ( 'NONE', ( #1100, #29003, #121747, #78127 ) ) ;
#116247=CIRCLE ( 'NONE', #11987, 0.1000000000000002554 ) ;
#116248=ORIENTED_EDGE ( 'NONE', *, *, #64794, .F. ) ;
#116250=DIRECTION ( 'NONE',  ( 0.000000000000000000, -0.000000000000000000, 1.000000000000000000 ) ) ;
#116251=CARTESIAN_POINT ( 'NONE',  ( -0.2000000000000347888, 2.500000000000000000, 0.3464101615137758494 ) ) ;
#116252=CARTESIAN_POINT ( 'NONE',  ( 13.09999999999989839, 2.500000000000000000, -0.3464101615137783474 ) ) ;
#116253=EDGE_LOOP ( 'NONE', ( #52968, #117408, #104013, #37614 ) ) ;
#116254=CIRCLE ( 'NONE', #41075, 0.1000000000000002554 ) ;
#116255=CIRCLE ( 'NONE', #22295, 0.1000000000000002554 ) ;
#116256=DIRECTION ( 'NONE',  ( 0.000000000000000000, 1.000000000000000000, 0.000000000000000000 ) ) ;
#116257=VECTOR ( 'NONE', #49769, 1000.000000000000000 ) ;
#116258=CARTESIAN_POINT ( 'NONE',  ( -11.25000000000000000, 2.500000000000000000, -2.757883832488650100 ) ) ;
#116260=DIRECTION ( 'NONE',  ( 0.000000000000000000, -0.9999939076577903929, 0.003490651415223739937 ) ) ;
#116261=DIRECTION ( 'NONE',  ( 0.000000000000000000, 1.000000000000000000, 0.000000000000000000 ) ) ;
#116262=ORIENTED_EDGE ( 'NONE', *, *, #15276, .F. ) ;
#116263=CARTESIAN_POINT ( 'NONE',  ( 6.249999999999928946, 2.500000000000000000, 2.857883832488649301 ) ) ;
#116264=VECTOR ( 'NONE', #16217, 1000.000000000000000 ) ;
#116265=VERTEX_POINT ( 'NONE', #112134 ) ;
#116266=AXIS2_PLACEMENT_3D ( 'NONE', #98720, #30664, #110487 ) ;
#116268=VERTEX_POINT ( 'NONE', #101669 ) ;
#116269=PLANE ( 'NONE',  #55138 ) ;
#116270=CARTESIAN_POINT ( 'NONE',  ( 9.399999999999918643, 12.50000000000000000, 0.2813168883297362810 ) ) ;
#116271=CARTESIAN_POINT ( 'NONE',  ( -11.04999999999999893, 12.50000000000000000, 1.818653347947321475 ) ) ;
#116272=ORIENTED_EDGE ( 'NONE', *, *, #15700, .T. ) ;
#116273=EDGE_LOOP ( 'NONE', ( #5104, #115356, #56707, #86982 ) ) ;
#116274=DIRECTION ( 'NONE',  ( -0.000000000000000000, 1.000000000000000000, -0.000000000000000000 ) ) ;
#116275=EDGE_CURVE ( 'NONE', #7829, #7349, #100375, .T. ) ;
#116276=DIRECTION ( 'NONE',  ( 0.000000000000000000, -0.000000000000000000, 1.000000000000000000 ) ) ;
#116277=DIRECTION ( 'NONE',  ( 0.000000000000000000, -0.9999939076577903929, 0.003490651415223739937 ) ) ;
#116278=ORIENTED_EDGE ( 'NONE', *, *, #29123, .T. ) ;
#116279=ORIENTED_EDGE ( 'NONE', *, *, #51625, .T. ) ;
#116280=DIRECTION ( 'NONE',  ( 0.000000000000000000, 1.000000000000000000, 0.000000000000000000 ) ) ;
#116281=ORIENTED_EDGE ( 'NONE', *, *, #82669, .F. ) ;
#116282=FACE_OUTER_BOUND ( 'NONE', #73638, .T. ) ;
#116283=CARTESIAN_POINT ( 'NONE',  ( -6.249999999999981348, 2.500000000000000000, 6.495190528383297135 ) ) ;
#116284=ORIENTED_EDGE ( 'NONE', *, *, #5673, .F. ) ;
#116285=LINE ( 'NONE', #26634, #2189 ) ;
#116286=PLANE ( 'NONE',  #119386 ) ;
#116287=DIRECTION ( 'NONE',  ( 0.000000000000000000, -0.000000000000000000, 1.000000000000000000 ) ) ;
#116288=EDGE_CURVE ( 'NONE', #40954, #32314, #15772, .T. ) ;
#116289=LINE ( 'NONE', #37751, #54261 ) ;
#116290=VERTEX_POINT ( 'NONE', #40832 ) ;
#116291=CARTESIAN_POINT ( 'NONE',  ( 4.149999999999941735, 12.50000000000000000, -2.922977105672691422 ) ) ;
#116292=AXIS2_PLACEMENT_3D ( 'NONE', #128372, #38709, #97593 ) ;
#116293=VECTOR ( 'NONE', #127611, 1000.000000000000000 ) ;
#116294=DIRECTION ( 'NONE',  ( -0.000000000000000000, -1.000000000000000000, -0.000000000000000000 ) ) ;
#116295=VERTEX_POINT ( 'NONE', #52556 ) ;
#116296=ORIENTED_EDGE ( 'NONE', *, *, #22761, .T. ) ;
#116298=CARTESIAN_POINT ( 'NONE',  ( 11.44999999999990514, 12.50000000000000000, 2.511473670974873507 ) ) ;
#116299=CARTESIAN_POINT ( 'NONE',  ( 11.64999999999990443, 2.500000000000000000, 2.757883832488649656 ) ) ;
#116300=CARTESIAN_POINT ( 'NONE',  ( 14.54999999999989235, 2.500000000000000000, -2.165063509461101710 ) ) ;
#116301=DIRECTION ( 'NONE',  ( 0.000000000000000000, 0.000000000000000000, 1.000000000000000000 ) ) ;
#116302=CONICAL_SURFACE ( 'NONE', #118456, 0.1000000000000002554, 0.003490658503988666988 ) ;
#116303=DIRECTION ( 'NONE',  ( 0.000000000000000000, 0.000000000000000000, 1.000000000000000000 ) ) ;
#116304=AXIS2_PLACEMENT_3D ( 'NONE', #101258, #29307, #90794 ) ;
#116305=CARTESIAN_POINT ( 'NONE',  ( 11.84999999999990372, 12.50000000000000000, -6.148780366869526226 ) ) ;
#116306=CARTESIAN_POINT ( 'NONE',  ( 2.699999999999945555, 2.500000000000000000, 4.083716857408420609 ) ) ;
#116307=CARTESIAN_POINT ( 'NONE',  ( 12.94999999999989981, 12.50000000000000000, -2.230156782645139391 ) ) ;
#116308=CARTESIAN_POINT ( 'NONE',  ( -13.09999999999999254, 2.500000000000000000, -3.883716857408423984 ) ) ;
#116309=AXIS2_PLACEMENT_3D ( 'NONE', #112639, #81866, #52417 ) ;
#116310=AXIS2_PLACEMENT_3D ( 'NONE', #51833, #31545, #102221 ) ;
#116311=EDGE_LOOP ( 'NONE', ( #36974, #63134, #98039, #111574 ) ) ;
#116312=AXIS2_PLACEMENT_3D ( 'NONE', #84414, #42582, #113885 ) ;
#116313=ADVANCED_FACE ( 'NONE', ( #1515 ), #84741, .T. ) ;
#116315=DIRECTION ( 'NONE',  ( 0.000000000000000000, 0.000000000000000000, -1.000000000000000000 ) ) ;
#116317=DIRECTION ( 'NONE',  ( -4.274815082592931898E-19, -0.9999939076577903929, -0.003490651415223739937 ) ) ;
#116318=DIRECTION ( 'NONE',  ( 0.000000000000000000, 0.000000000000000000, 1.000000000000000000 ) ) ;
#116321=ORIENTED_EDGE ( 'NONE', *, *, #78534, .T. ) ;
#116322=DIRECTION ( 'NONE',  ( 0.000000000000000000, 0.000000000000000000, 1.000000000000000000 ) ) ;
#116324=DIRECTION ( 'NONE',  ( -4.274815082592931898E-19, -0.9999939076577903929, -0.003490651415223739937 ) ) ;
#116325=ORIENTED_EDGE ( 'NONE', *, *, #21276, .F. ) ;
#116326=EDGE_CURVE ( 'NONE', #88048, #4024, #5306, .T. ) ;
#116327=EDGE_CURVE ( 'NONE', #112183, #18217, #61781, .T. ) ;
#116328=ADVANCED_FACE ( 'NONE', ( #13263 ), #53218, .T. ) ;
#116329=ADVANCED_FACE ( 'NONE', ( #113414 ), #3460, .T. ) ;
#116330=CIRCLE ( 'NONE', #36936, 0.06509327318403745899 ) ;
#116331=ADVANCED_FACE ( 'NONE', ( #94403 ), #44037, .T. ) ;
#116332=CARTESIAN_POINT ( 'NONE',  ( 8.749999999999953815, 2.500000000000000000, 6.595190528383296780 ) ) ;
#116333=VERTEX_POINT ( 'NONE', #74785 ) ;
#116334=CIRCLE ( 'NONE', #20504, 0.1000000000000002554 ) ;
#116335=AXIS2_PLACEMENT_3D ( 'NONE', #7528, #50070, #89960 ) ;
#116336=VERTEX_POINT ( 'NONE', #95069 ) ;
#116337=ORIENTED_EDGE ( 'NONE', *, *, #74711, .F. ) ;
#116338=ORIENTED_EDGE ( 'NONE', *, *, #37363, .F. ) ;
#116339=DIRECTION ( 'NONE',  ( 0.000000000000000000, 0.000000000000000000, 1.000000000000000000 ) ) ;
#116340=EDGE_CURVE ( 'NONE', #83167, #47460, #23756, .T. ) ;
#116341=AXIS2_PLACEMENT_3D ( 'NONE', #36074, #115914, #16398 ) ;
#116342=DIRECTION ( 'NONE',  ( 0.000000000000000000, 1.000000000000000000, 0.000000000000000000 ) ) ;
#116343=CARTESIAN_POINT ( 'NONE',  ( -9.400000000000009237, 2.500000000000000000, -3.983716857408421852 ) ) ;
#116344=EDGE_CURVE ( 'NONE', #83303, #104829, #55500, .T. ) ;
#116345=DIRECTION ( 'NONE',  ( 0.000000000000000000, 0.000000000000000000, 1.000000000000000000 ) ) ;
#116346=ADVANCED_FACE ( 'NONE', ( #114689 ), #22067, .T. ) ;
#116347=ORIENTED_EDGE ( 'NONE', *, *, #81028, .F. ) ;
#116348=CIRCLE ( 'NONE', #15993, 0.1000000000000002554 ) ;
#116349=DIRECTION ( 'NONE',  ( 0.000000000000000000, 1.000000000000000000, 0.000000000000000000 ) ) ;
#116350=ORIENTED_EDGE ( 'NONE', *, *, #51280, .T. ) ;
#116351=CARTESIAN_POINT ( 'NONE',  ( 81.97673105564510365, -3.779183769821120809, -6.223416305047164698 ) ) ;
#116352=FACE_OUTER_BOUND ( 'NONE', #111541, .T. ) ;
#116353=CARTESIAN_POINT ( 'NONE',  ( 4.799999999999937650, 2.500000000000000000, -3.983716857408426293 ) ) ;
#116354=CARTESIAN_POINT ( 'NONE',  ( 20.80581321129229977, -0.6997403544481954896, 4.161084241360361702 ) ) ;
#116355=AXIS2_PLACEMENT_3D ( 'NONE', #49171, #9221, #9869 ) ;
#116356=AXIS2_PLACEMENT_3D ( 'NONE', #95774, #98338, #88520 ) ;
#116357=EDGE_LOOP ( 'NONE', ( #105562, #18779, #115905, #96424 ) ) ;
#116358=VECTOR ( 'NONE', #49506, 1000.000000000000000 ) ;
#116359=CONICAL_SURFACE ( 'NONE', #74608, 0.1000000000000000056, 0.003490658503988666988 ) ;
#116360=ORIENTED_EDGE ( 'NONE', *, *, #37474, .F. ) ;
#116362=CARTESIAN_POINT ( 'NONE',  ( 11.89999999999990798, 12.50000000000000000, -3.918623584224389056 ) ) ;
#116363=DIRECTION ( 'NONE',  ( 0.000000000000000000, 1.000000000000000000, 0.000000000000000000 ) ) ;
#116364=DIRECTION ( 'NONE',  ( 0.000000000000000000, 0.000000000000000000, 1.000000000000000000 ) ) ;
#116365=FACE_BOUND ( 'NONE', #23367, .T. ) ;
#116366=DIRECTION ( 'NONE',  ( 0.000000000000000000, 0.000000000000000000, 1.000000000000000000 ) ) ;
#116367=CARTESIAN_POINT ( 'NONE',  ( -10.60000000000000142, 2.500000000000000000, 0.3464101615137736845 ) ) ;
#116368=CARTESIAN_POINT ( 'NONE',  ( -11.64999999999999680, 12.50000000000000000, -7.188010851410850499 ) ) ;
#116369=DIRECTION ( 'NONE',  ( 0.000000000000000000, 1.000000000000000000, 0.000000000000000000 ) ) ;
#116370=B_SPLINE_CURVE_WITH_KNOTS ( 'NONE', 3,
 ( #48030, #118035, #67641, #19171, #87912, #27092, #89227, #88579, #9382, #36917, #116739, #108217, #28385, #57187, #17233, #107582, #49330, #17900 ),
 .UNSPECIFIED., .F., .F.,
 ( 4, 2, 2, 2, 2, 2, 2, 2, 4 ),
 ( -1.046607274944427702E-05, 0.0004931538261984684448, 0.0009967737251463811531, 0.002004013523042207003, 0.002507633421990117760, 0.002759443371464072054, 0.003011253320938025915, 0.003514873219885932334, 0.004018493118833838321 ),
 .UNSPECIFIED. ) ;
#116372=EDGE_CURVE ( 'NONE', #127574, #31579, #113991, .T. ) ;
#116373=DIRECTION ( 'NONE',  ( -0.000000000000000000, -1.000000000000000000, -0.000000000000000000 ) ) ;
#116374=DIRECTION ( 'NONE',  ( 0.000000000000000000, -0.000000000000000000, 1.000000000000000000 ) ) ;
#116375=DIRECTION ( 'NONE',  ( 0.000000000000000000, -0.000000000000000000, 1.000000000000000000 ) ) ;
#116376=ORIENTED_EDGE ( 'NONE', *, *, #87841, .F. ) ;
#116377=ORIENTED_EDGE ( 'NONE', *, *, #125839, .T. ) ;
#116378=ORIENTED_EDGE ( 'NONE', *, *, #79153, .T. ) ;
#116379=ORIENTED_EDGE ( 'NONE', *, *, #101279, .F. ) ;
#116380=DIRECTION ( 'NONE',  ( 0.000000000000000000, 0.000000000000000000, 1.000000000000000000 ) ) ;
#116381=EDGE_CURVE ( 'NONE', #75694, #95476, #84460, .T. ) ;
#116382=FACE_BOUND ( 'NONE', #38105, .T. ) ;
#116383=CARTESIAN_POINT ( 'NONE',  ( 8.749999999999918288, 12.50000000000000000, -1.537336459617587581 ) ) ;
#116384=CARTESIAN_POINT ( 'NONE',  ( 4.349999999999941025, 2.500000000000000000, -1.818653347947326138 ) ) ;
#116385=ADVANCED_FACE ( 'NONE', ( #93140 ), #28025, .T. ) ;
#116386=CIRCLE ( 'NONE', #62031, 0.1000000000000002554 ) ;
#116387=AXIS2_PLACEMENT_3D ( 'NONE', #50666, #18624, #118109 ) ;
#116388=EDGE_CURVE ( 'NONE', #34384, #5489, #123242, .T. ) ;
#116389=ORIENTED_EDGE ( 'NONE', *, *, #128761, .F. ) ;
#116390=DIRECTION ( 'NONE',  ( 0.000000000000000000, 0.000000000000000000, -1.000000000000000000 ) ) ;
#116391=LINE ( 'NONE', #107224, #104323 ) ;
#116392=ORIENTED_EDGE ( 'NONE', *, *, #33352, .T. ) ;
#116393=CARTESIAN_POINT ( 'NONE',  ( 10.44999999999991047, 2.500000000000000000, -6.395190528383301931 ) ) ;
#116394=DIRECTION ( 'NONE',  ( 0.000000000000000000, 0.000000000000000000, 1.000000000000000000 ) ) ;
#116395=ADVANCED_FACE ( 'NONE', ( #104862 ), #68014, .T. ) ;
#116396=VECTOR ( 'NONE', #120390, 1000.000000000000000 ) ;
#116397=ORIENTED_EDGE ( 'NONE', *, *, #48543, .F. ) ;
#116398=FACE_OUTER_BOUND ( 'NONE', #46864, .T. ) ;
#116399=CARTESIAN_POINT ( 'NONE',  ( 6.649999999999931077, 2.500000000000000000, -6.595190528383302109 ) ) ;
#116400=CONICAL_SURFACE ( 'NONE', #26627, 0.09999999999999999167, 0.003490658503988666988 ) ;
#116401=VECTOR ( 'NONE', #113317, 1000.000000000000000 ) ;
#116402=ORIENTED_EDGE ( 'NONE', *, *, #125271, .F. ) ;
#116403=AXIS2_PLACEMENT_3D ( 'NONE', #38848, #118653, #86617 ) ;
#116404=CARTESIAN_POINT ( 'NONE',  ( 5.649999999999936406, 2.500000000000000000, -6.248780366869526759 ) ) ;
#116405=PLANE ( 'NONE',  #37291 ) ;
#116406=ORIENTED_EDGE ( 'NONE', *, *, #1697, .F. ) ;
#116407=DIRECTION ( 'NONE',  ( 0.000000000000000000, -0.9999939076577903929, 0.003490651415223739937 ) ) ;
#116408=ORIENTED_EDGE ( 'NONE', *, *, #5774, .T. ) ;
#116409=ORIENTED_EDGE ( 'NONE', *, *, #70945, .F. ) ;
#116410=DIRECTION ( 'NONE',  ( -0.000000000000000000, -1.000000000000000000, -0.000000000000000000 ) ) ;
#116411=ADVANCED_FACE ( 'NONE', ( #115311 ), #63822, .T. ) ;
#116412=ORIENTED_EDGE ( 'NONE', *, *, #16753, .F. ) ;
#116413=DIRECTION ( 'NONE',  ( 0.000000000000000000, 0.000000000000000000, 1.000000000000000000 ) ) ;
#116414=DIRECTION ( 'NONE',  ( 0.000000000000000000, 0.000000000000000000, 1.000000000000000000 ) ) ;
#116415=VERTEX_POINT ( 'NONE', #4092 ) ;
#116416=CARTESIAN_POINT ( 'NONE',  ( -1.850000000000033840, 2.500000000000000000, 1.818653347947321475 ) ) ;
#116417=CARTESIAN_POINT ( 'NONE',  ( -10.84999999999999964, 2.500000000000000000, 2.857883832488649301 ) ) ;
#116418=CARTESIAN_POINT ( 'NONE',  ( 8.299999999999922551, 2.500000000000000000, -4.230127018922201998 ) ) ;
#116419=DIRECTION ( 'NONE',  ( 0.000000000000000000, 1.000000000000000000, 0.000000000000000000 ) ) ;
#116420=DIRECTION ( 'NONE',  ( 0.000000000000000000, 0.000000000000000000, -1.000000000000000000 ) ) ;
#116421=AXIS2_PLACEMENT_3D ( 'NONE', #45611, #106445, #14182 ) ;
#116422=CARTESIAN_POINT ( 'NONE',  ( -0.4500000000000397571, 2.500000000000000000, -2.165063509461101710 ) ) ;
#116423=AXIS2_PLACEMENT_3D ( 'NONE', #86309, #36608, #95502 ) ;
#116424=CIRCLE ( 'NONE', #11973, 0.09999999999999982514 ) ;
#116425=VERTEX_POINT ( 'NONE', #55142 ) ;
#116426=EDGE_LOOP ( 'NONE', ( #45299, #85670 ) ) ;
#116428=CIRCLE ( 'NONE', #39104, 0.06509327318403745899 ) ;
#116429=EDGE_CURVE ( 'NONE', #102116, #120297, #101475, .T. ) ;
#116430=CARTESIAN_POINT ( 'NONE',  ( -6.450000000000019718, 12.50000000000000000, -6.213873640053564351 ) ) ;
#116431=LINE ( 'NONE', #94222, #66904 ) ;
#116432=VERTEX_POINT ( 'NONE', #104238 ) ;
#116433=VERTEX_POINT ( 'NONE', #76070 ) ;
#116434=EDGE_LOOP ( 'NONE', ( #98648, #18851, #10617, #67385 ) ) ;
#116435=DIRECTION ( 'NONE',  ( -0.000000000000000000, 1.000000000000000000, -0.000000000000000000 ) ) ;
#116436=CONICAL_SURFACE ( 'NONE', #120560, 0.1000000000000000472, 0.003490658503988666988 ) ;
#116437=AXIS2_PLACEMENT_3D ( 'NONE', #111744, #83585, #22093 ) ;
#116438=FACE_OUTER_BOUND ( 'NONE', #99254, .T. ) ;
#116439=DIRECTION ( 'NONE',  ( 0.000000000000000000, 0.000000000000000000, 1.000000000000000000 ) ) ;
#116440=CIRCLE ( 'NONE', #62092, 0.09999999999999999167 ) ;
#116442=FACE_OUTER_BOUND ( 'NONE', #25422, .T. ) ;
#116443=DIRECTION ( 'NONE',  ( 0.000000000000000000, 0.000000000000000000, 1.000000000000000000 ) ) ;
#116444=CARTESIAN_POINT ( 'NONE',  ( 10.79999999999991367, 2.500000000000000000, -2.385244779468109755E-15 ) ) ;
#116445=CARTESIAN_POINT ( 'NONE',  ( -8.750000000000010658, 2.500000000000000000, -1.372243186433550033 ) ) ;
#116446=DIRECTION ( 'NONE',  ( 0.000000000000000000, 0.000000000000000000, 1.000000000000000000 ) ) ;
#116447=AXIS2_PLACEMENT_3D ( 'NONE', #5823, #85038, #115793 ) ;
#116448=ADVANCED_FACE ( 'NONE', ( #14552 ), #118191, .T. ) ;
#116449=DIRECTION ( 'NONE',  ( 0.000000000000000000, -0.9999939076577903929, 0.003490651415223739937 ) ) ;
#116450=AXIS2_PLACEMENT_3D ( 'NONE', #93688, #13823, #54400 ) ;
#116451=VERTEX_POINT ( 'NONE', #106178 ) ;
#116452=AXIS2_PLACEMENT_3D ( 'NONE', #129213, #128567, #9412 ) ;
#116453=AXIS2_PLACEMENT_3D ( 'NONE', #121559, #41747, #113037 ) ;
#116454=DIRECTION ( 'NONE',  ( -0.000000000000000000, 1.000000000000000000, -0.000000000000000000 ) ) ;
#116455=ORIENTED_EDGE ( 'NONE', *, *, #65947, .T. ) ;
#116456=ORIENTED_EDGE ( 'NONE', *, *, #73254, .F. ) ;
#116457=FACE_OUTER_BOUND ( 'NONE', #90381, .T. ) ;
#116458=CARTESIAN_POINT ( 'NONE',  ( 3.149999999999942624, 2.500000000000000000, 6.841600689897072485 ) ) ;
#116459=CARTESIAN_POINT ( 'NONE',  ( 12.49999999999990585, 2.500000000000000000, -4.922947341949753586 ) ) ;
#116460=CARTESIAN_POINT ( 'NONE',  ( -4.999999999999986677, 2.500000000000000000, 0.09999999999999772959 ) ) ;
#116461=FACE_OUTER_BOUND ( 'NONE', #61368, .T. ) ;
#116462=CARTESIAN_POINT ( 'NONE',  ( -7.700000000000016165, 12.50000000000000000, -3.983716857408426293 ) ) ;
#116463=FACE_OUTER_BOUND ( 'NONE', #67777, .T. ) ;
#116464=VERTEX_POINT ( 'NONE', #15845 ) ;
#116465=FACE_OUTER_BOUND ( 'NONE', #72424, .T. ) ;
#116466=CIRCLE ( 'NONE', #106104, 0.1000000000000002554 ) ;
#116467=FACE_OUTER_BOUND ( 'NONE', #90760, .T. ) ;
#116468=ORIENTED_EDGE ( 'NONE', *, *, #51166, .T. ) ;
#116469=EDGE_LOOP ( 'NONE', ( #95713, #17188 ) ) ;
#116470=EDGE_CURVE ( 'NONE', #28339, #82935, #47107, .T. ) ;
#116471=ORIENTED_EDGE ( 'NONE', *, *, #79630, .T. ) ;
#116472=ORIENTED_EDGE ( 'NONE', *, *, #115648, .F. ) ;
#116473=ORIENTED_EDGE ( 'NONE', *, *, #96261, .F. ) ;
#116475=DIRECTION ( 'NONE',  ( -0.000000000000000000, -1.000000000000000000, -0.000000000000000000 ) ) ;
#116476=ADVANCED_FACE ( 'NONE', ( #16478 ), #43406, .T. ) ;
#116477=EDGE_LOOP ( 'NONE', ( #113212, #28737 ) ) ;
#116478=AXIS2_PLACEMENT_3D ( 'NONE', #53650, #3899, #43854 ) ;
#116479=DIRECTION ( 'NONE',  ( -0.000000000000000000, 1.000000000000000000, -0.000000000000000000 ) ) ;
#116480=AXIS2_PLACEMENT_3D ( 'NONE', #112169, #63715, #61793 ) ;
#116481=CARTESIAN_POINT ( 'NONE',  ( -11.89999999999999503, 2.500000000000000000, 4.776537180435972196 ) ) ;
#116482=DIRECTION ( 'NONE',  ( 0.000000000000000000, 0.000000000000000000, 1.000000000000000000 ) ) ;
#116483=ORIENTED_EDGE ( 'NONE', *, *, #22622, .F. ) ;
#116484=EDGE_CURVE ( 'NONE', #9001, #37856, #56416, .T. ) ;
#116485=EDGE_CURVE ( 'NONE', #32461, #10213, #37445, .T. ) ;
#116486=ADVANCED_FACE ( 'NONE', ( #117912 ), #48545, .T. ) ;
#116487=CARTESIAN_POINT ( 'NONE',  ( -0.8500000000000390576, 2.500000000000000000, -2.065063509461102065 ) ) ;
#116488=EDGE_CURVE ( 'NONE', #45295, #32793, #109791, .T. ) ;
#116489=AXIS2_PLACEMENT_3D ( 'NONE', #59403, #110400, #128122 ) ;
#116490=AXIS2_PLACEMENT_3D ( 'NONE', #60175, #100086, #88974 ) ;
#116491=DIRECTION ( 'NONE',  ( -4.274815082592931898E-19, -0.9999939076577903929, -0.003490651415223739937 ) ) ;
#116492=ORIENTED_EDGE ( 'NONE', *, *, #97851, .T. ) ;
#116493=CONICAL_SURFACE ( 'NONE', #91457, 0.09999999999999982514, 0.003490658503988666988 ) ;
#116494=VERTEX_POINT ( 'NONE', #127113 ) ;
#116495=EDGE_CURVE ( 'NONE', #123810, #65564, #11291, .T. ) ;
#116496=EDGE_LOOP ( 'NONE', ( #12874, #72405 ) ) ;
#116497=DIRECTION ( 'NONE',  ( -0.000000000000000000, -1.000000000000000000, -0.000000000000000000 ) ) ;
#116498=EDGE_CURVE ( 'NONE', #124819, #50249, #116040, .T. ) ;
#116499=ADVANCED_FACE ( 'NONE', ( #47264 ), #26973, .T. ) ;
#116500=AXIS2_PLACEMENT_3D ( 'NONE', #95462, #115735, #65339 ) ;
#116501=DIRECTION ( 'NONE',  ( 0.000000000000000000, 0.000000000000000000, -1.000000000000000000 ) ) ;
#116502=EDGE_CURVE ( 'NONE', #25999, #92156, #96333, .T. ) ;
#116503=AXIS2_PLACEMENT_3D ( 'NONE', #32881, #34817, #14482 ) ;
#116504=EDGE_CURVE ( 'NONE', #3741, #107010, #126514, .T. ) ;
#116505=ORIENTED_EDGE ( 'NONE', *, *, #39922, .T. ) ;
#116506=CARTESIAN_POINT ( 'NONE',  ( -1.850000000000033396, 2.500000000000000000, -2.511473670974877948 ) ) ;
#116507=DIRECTION ( 'NONE',  ( -4.274815082592931898E-19, -0.9999939076577903929, -0.003490651415223739937 ) ) ;
#116508=DIRECTION ( 'NONE',  ( 0.000000000000000000, 1.000000000000000000, 0.000000000000000000 ) ) ;
#116509=DIRECTION ( 'NONE',  ( -4.274815082592931898E-19, -0.9999939076577903929, -0.003490651415223739937 ) ) ;
#116511=ORIENTED_EDGE ( 'NONE', *, *, #96520, .T. ) ;
#116512=CARTESIAN_POINT ( 'NONE',  ( 14.34999999999989306, 12.50000000000000000, -2.446380397790840266 ) ) ;
#116513=CONICAL_SURFACE ( 'NONE', #114461, 0.09999999999999982514, 0.003490658503988666988 ) ;
#116514=VERTEX_POINT ( 'NONE', #17777 ) ;
#116515=EDGE_LOOP ( 'NONE', ( #115119, #49094, #110332, #9956 ) ) ;
#116516=EDGE_LOOP ( 'NONE', ( #50243, #129516 ) ) ;
#116517=CARTESIAN_POINT ( 'NONE',  ( 11.24999999999991118, 2.500000000000000000, 5.702370205355745014 ) ) ;
#116518=FACE_BOUND ( 'NONE', #8970, .T. ) ;
#116519=CIRCLE ( 'NONE', #14106, 0.1000000000000000472 ) ;
#116521=DIRECTION ( 'NONE',  ( 0.000000000000000000, 1.000000000000000000, 0.000000000000000000 ) ) ;
#116522=CIRCLE ( 'NONE', #47590, 0.1000000000000000056 ) ;
#116523=CARTESIAN_POINT ( 'NONE',  ( 0.6499999999999543920, 2.500000000000000000, 6.741600689897071952 ) ) ;
#116524=CIRCLE ( 'NONE', #127008, 0.06509327318403745899 ) ;
#116525=ORIENTED_EDGE ( 'NONE', *, *, #59202, .F. ) ;
#116526=CARTESIAN_POINT ( 'NONE',  ( 13.09999999999990195, 12.50000000000000000, 4.048810130592458201 ) ) ;
#116527=DIRECTION ( 'NONE',  ( -0.000000000000000000, 1.000000000000000000, -0.000000000000000000 ) ) ;
#116528=AXIS2_PLACEMENT_3D ( 'NONE', #1622, #29177, #50732 ) ;
#116529=CARTESIAN_POINT ( 'NONE',  ( 16.87640210516335415, 2.500000000000000000, 4.436424697255048955 ) ) ;
#116530=AXIS2_PLACEMENT_3D ( 'NONE', #58637, #109662, #8856 ) ;
#116531=DIRECTION ( 'NONE',  ( 0.000000000000000000, 0.000000000000000000, -1.000000000000000000 ) ) ;
#116532=EDGE_LOOP ( 'NONE', ( #26980, #25867 ) ) ;
#116533=DIRECTION ( 'NONE',  ( -0.000000000000000000, 1.000000000000000000, -0.000000000000000000 ) ) ;
#116534=AXIS2_PLACEMENT_3D ( 'NONE', #41484, #33427, #29078 ) ;
#116535=CIRCLE ( 'NONE', #70478, 0.06509327318403745899 ) ;
#116536=CARTESIAN_POINT ( 'NONE',  ( 1.699999999999951994, 2.500000000000000000, -4.230127018922201998 ) ) ;
#116537=ORIENTED_EDGE ( 'NONE', *, *, #48069, .T. ) ;
#116538=DIRECTION ( 'NONE',  ( 0.000000000000000000, 1.000000000000000000, 0.000000000000000000 ) ) ;
#116539=CIRCLE ( 'NONE', #101884, 0.1000000000000000472 ) ;
#116540=DIRECTION ( 'NONE',  ( -0.000000000000000000, 1.000000000000000000, -0.000000000000000000 ) ) ;
#116541=FACE_BOUND ( 'NONE', #119227, .T. ) ;
#116542=CARTESIAN_POINT ( 'NONE',  ( 2.500000000000002220, -2.500000000000000000, -8.999999999999998224 ) ) ;
#116543=EDGE_CURVE ( 'NONE', #117070, #71126, #103528, .T. ) ;
#116545=ORIENTED_EDGE ( 'NONE', *, *, #128060, .F. ) ;
#116546=DIRECTION ( 'NONE',  ( -0.000000000000000000, -1.000000000000000000, -0.000000000000000000 ) ) ;
#116548=EDGE_LOOP ( 'NONE', ( #90857, #97347 ) ) ;
#116549=ORIENTED_EDGE ( 'NONE', *, *, #9115, .F. ) ;
#116550=FACE_OUTER_BOUND ( 'NONE', #68549, .T. ) ;
#116552=VERTEX_POINT ( 'NONE', #18434 ) ;
#116553=DIRECTION ( 'NONE',  ( 0.000000000000000000, 0.000000000000000000, 1.000000000000000000 ) ) ;
#116554=FACE_OUTER_BOUND ( 'NONE', #106534, .T. ) ;
#116555=EDGE_CURVE ( 'NONE', #48757, #109936, #116625, .T. ) ;
#116556=CARTESIAN_POINT ( 'NONE',  ( 7.499999999999961808, 2.500000000000000000, -4.330127018922201643 ) ) ;
#116557=DIRECTION ( 'NONE',  ( 0.000000000000000000, 0.000000000000000000, 1.000000000000000000 ) ) ;
#116559=ORIENTED_EDGE ( 'NONE', *, *, #27340, .F. ) ;
#116560=CARTESIAN_POINT ( 'NONE',  ( 5.849999999999933920, 2.500000000000000000, 6.495190528383297135 ) ) ;
#116561=DIRECTION ( 'NONE',  ( -0.000000000000000000, -1.000000000000000000, -0.000000000000000000 ) ) ;
#116562=DIRECTION ( 'NONE',  ( 0.000000000000000000, 0.000000000000000000, -1.000000000000000000 ) ) ;
#116563=CARTESIAN_POINT ( 'NONE',  ( 21.25104915411511897, 0.2454763298552203044, -4.189301388123448433 ) ) ;
#116564=ORIENTED_EDGE ( 'NONE', *, *, #88571, .F. ) ;
#116565=DIRECTION ( 'NONE',  ( -0.000000000000000000, 1.000000000000000000, -0.000000000000000000 ) ) ;
#116566=ORIENTED_EDGE ( 'NONE', *, *, #117412, .F. ) ;
#116567=CARTESIAN_POINT ( 'NONE',  ( -3.350000000000032507, 12.50000000000000000, -6.430097255199264339 ) ) ;
#116568=DIRECTION ( 'NONE',  ( 0.000000000000000000, 1.000000000000000000, 0.000000000000000000 ) ) ;
#116569=VERTEX_POINT ( 'NONE', #11011 ) ;
#116570=DIRECTION ( 'NONE',  ( 0.000000000000000000, 0.000000000000000000, 1.000000000000000000 ) ) ;
#116571=FACE_OUTER_BOUND ( 'NONE', #11621, .T. ) ;
#116572=AXIS2_PLACEMENT_3D ( 'NONE', #39531, #99719, #107597 ) ;
#116573=CARTESIAN_POINT ( 'NONE',  ( 9.349999999999916156, 2.500000000000000000, 6.741600689897071952 ) ) ;
#116574=AXIS2_PLACEMENT_3D ( 'NONE', #22361, #91077, #43287 ) ;
#116575=DIRECTION ( 'NONE',  ( -4.274815082592931898E-19, -0.9999939076577903929, -0.003490651415223739937 ) ) ;
#116576=ORIENTED_EDGE ( 'NONE', *, *, #58245, .F. ) ;
#116577=CARTESIAN_POINT ( 'NONE',  ( -15.59999999999998010, 12.50000000000000000, 0.2813168883297385570 ) ) ;
#116578=DIRECTION ( 'NONE',  ( -4.274815082592931898E-19, -0.9999939076577903929, -0.003490651415223739937 ) ) ;
#116579=FACE_OUTER_BOUND ( 'NONE', #27618, .T. ) ;
#116580=CARTESIAN_POINT ( 'NONE',  ( 3.949999999999939782, 2.500000000000000000, 2.611473670974873151 ) ) ;
#116582=AXIS2_PLACEMENT_3D ( 'NONE', #116774, #6795, #46764 ) ;
#116583=ADVANCED_FACE ( 'NONE', ( #38076 ), #109601, .T. ) ;
#116584=VERTEX_POINT ( 'NONE', #67509 ) ;
#116585=CIRCLE ( 'NONE', #83450, 0.06509327318403745899 ) ;
#116586=ORIENTED_EDGE ( 'NONE', *, *, #14187, .F. ) ;
#116587=CARTESIAN_POINT ( 'NONE',  ( 7.949999999999922018, 12.50000000000000000, 6.495190528383297135 ) ) ;
#116588=ORIENTED_EDGE ( 'NONE', *, *, #50577, .T. ) ;
#116589=DIRECTION ( 'NONE',  ( 0.000000000000000000, 0.000000000000000000, -1.000000000000000000 ) ) ;
#116590=VERTEX_POINT ( 'NONE', #81071 ) ;
#116591=VERTEX_POINT ( 'NONE', #107457 ) ;
#116592=ORIENTED_EDGE ( 'NONE', *, *, #51226, .T. ) ;
#116593=DIRECTION ( 'NONE',  ( 0.000000000000000000, 0.000000000000000000, -1.000000000000000000 ) ) ;
#116594=AXIS2_PLACEMENT_3D ( 'NONE', #122535, #113344, #23683 ) ;
#116595=FACE_OUTER_BOUND ( 'NONE', #81125, .T. ) ;
#116596=CARTESIAN_POINT ( 'NONE',  ( -14.19999999999998685, 12.50000000000000000, -1.084202172485504434E-16 ) ) ;
#116598=FACE_OUTER_BOUND ( 'NONE', #16325, .T. ) ;
#116599=DIRECTION ( 'NONE',  ( 0.000000000000000000, 1.000000000000000000, 0.000000000000000000 ) ) ;
#116600=ADVANCED_FACE ( 'NONE', ( #66878 ), #21776, .T. ) ;
#116601=LINE ( 'NONE', #78643, #120798 ) ;
#116602=AXIS2_PLACEMENT_3D ( 'NONE', #129236, #57904, #99757 ) ;
#116603=ORIENTED_EDGE ( 'NONE', *, *, #49537, .F. ) ;
#116604=EDGE_CURVE ( 'NONE', #14341, #62130, #5021, .T. ) ;
#116605=FACE_OUTER_BOUND ( 'NONE', #34947, .T. ) ;
#116606=ORIENTED_EDGE ( 'NONE', *, *, #15969, .F. ) ;
#116607=AXIS2_PLACEMENT_3D ( 'NONE', #30909, #30268, #89805 ) ;
#116608=ORIENTED_EDGE ( 'NONE', *, *, #44334, .F. ) ;
#116609=ORIENTED_EDGE ( 'NONE', *, *, #91858, .F. ) ;
#116610=ORIENTED_EDGE ( 'NONE', *, *, #57203, .T. ) ;
#116611=DIRECTION ( 'NONE',  ( 0.000000000000000000, -0.000000000000000000, 1.000000000000000000 ) ) ;
#116613=EDGE_CURVE ( 'NONE', #119461, #86952, #70599, .T. ) ;
#116614=ORIENTED_EDGE ( 'NONE', *, *, #10966, .F. ) ;
#116615=AXIS2_PLACEMENT_3D ( 'NONE', #125925, #36296, #76205 ) ;
#116616=CONICAL_SURFACE ( 'NONE', #64386, 0.1000000000000002554, 0.003490658503988666988 ) ;
#116617=LINE ( 'NONE', #27581, #68609 ) ;
#116618=DIRECTION ( 'NONE',  ( -4.274815082592931898E-19, -0.9999939076577903929, -0.003490651415223739937 ) ) ;
#116620=CARTESIAN_POINT ( 'NONE',  ( -10.40000000000000213, 12.50000000000000000, -0.6928203230275541413 ) ) ;
#116621=DIRECTION ( 'NONE',  ( -0.000000000000000000, -1.000000000000000000, -0.000000000000000000 ) ) ;
#116622=LINE ( 'NONE', #108090, #13273 ) ;
#116623=ORIENTED_EDGE ( 'NONE', *, *, #103502, .F. ) ;
#116624=AXIS2_PLACEMENT_3D ( 'NONE', #119308, #88562, #99694 ) ;
#116625=LINE ( 'NONE', #87801, #34593 ) ;
#116626=CONICAL_SURFACE ( 'NONE', #126815, 0.09999999999999982514, 0.003490658503988666988 ) ;
#116627=ORIENTED_EDGE ( 'NONE', *, *, #95414, .F. ) ;
#116628=AXIS2_PLACEMENT_3D ( 'NONE', #76445, #88831, #122010 ) ;
#116629=DIRECTION ( 'NONE',  ( 0.000000000000000000, -0.000000000000000000, 1.000000000000000000 ) ) ;
#116630=EDGE_LOOP ( 'NONE', ( #7445, #78377, #122916, #126449 ) ) ;
#116631=DIRECTION ( 'NONE',  ( -0.000000000000000000, 1.000000000000000000, -0.000000000000000000 ) ) ;
#116632=ORIENTED_EDGE ( 'NONE', *, *, #63034, .F. ) ;
#116633=AXIS2_PLACEMENT_3D ( 'NONE', #75705, #6306, #43709 ) ;
#116634=EDGE_LOOP ( 'NONE', ( #30436, #46160 ) ) ;
#116635=CARTESIAN_POINT ( 'NONE',  ( -13.34999999999999076, 2.500000000000000000, 1.572243186433549544 ) ) ;
#116636=CARTESIAN_POINT ( 'NONE',  ( -0.2000000000000339284, 2.500000000000000000, -0.3464101615137759604 ) ) ;
#116637=ADVANCED_FACE ( 'NONE', ( #43739 ), #124264, .T. ) ;
#116638=AXIS2_PLACEMENT_3D ( 'NONE', #96983, #47256, #20847 ) ;
#116639=CIRCLE ( 'NONE', #125049, 0.1000000000000000472 ) ;
#116640=CARTESIAN_POINT ( 'NONE',  ( -0.8500000000000382805, 12.50000000000000000, -2.792790559304616504 ) ) ;
#116641=FACE_OUTER_BOUND ( 'NONE', #13550, .T. ) ;
#116642=DIRECTION ( 'NONE',  ( 0.000000000000000000, 1.000000000000000000, 0.000000000000000000 ) ) ;
#116643=ORIENTED_EDGE ( 'NONE', *, *, #97120, .T. ) ;
#116644=LINE ( 'NONE', #7976, #1761 ) ;
#116645=DIRECTION ( 'NONE',  ( -0.000000000000000000, 1.000000000000000000, -0.000000000000000000 ) ) ;
#116646=EDGE_CURVE ( 'NONE', #73230, #24288, #2479, .T. ) ;
#116647=DIRECTION ( 'NONE',  ( 0.000000000000000000, 0.000000000000000000, -1.000000000000000000 ) ) ;
#116648=CARTESIAN_POINT ( 'NONE',  ( -7.500000000000013323, 2.500000000000000000, 5.022947341949748790 ) ) ;
#116649=ADVANCED_FACE ( 'NONE', ( #22165 ), #11385, .T. ) ;
#116650=DIRECTION ( 'NONE',  ( -0.000000000000000000, -1.000000000000000000, -0.000000000000000000 ) ) ;
#116651=ORIENTED_EDGE ( 'NONE', *, *, #51846, .T. ) ;
#116652=EDGE_LOOP ( 'NONE', ( #89507, #24751 ) ) ;
#116653=EDGE_CURVE ( 'NONE', #55973, #108239, #111653, .T. ) ;
#116654=EDGE_CURVE ( 'NONE', #20003, #6508, #88661, .T. ) ;
#116655=CARTESIAN_POINT ( 'NONE',  ( 8.749999999999923617, 2.500000000000000000, -7.188010851410854052 ) ) ;
#116656=ADVANCED_FACE ( 'NONE', ( #103287 ), #3154, .T. ) ;
#116657=EDGE_LOOP ( 'NONE', ( #47906, #49831 ) ) ;
#116658=DIRECTION ( 'NONE',  ( 0.000000000000000000, -0.9999939076577903929, 0.003490651415223739937 ) ) ;
#116659=CARTESIAN_POINT ( 'NONE',  ( 4.349999999999936584, 12.50000000000000000, 6.148780366869520009 ) ) ;
#116660=EDGE_CURVE ( 'NONE', #6759, #42690, #61584, .T. ) ;
#116661=CIRCLE ( 'NONE', #18991, 0.06509327318403745899 ) ;
#116662=VERTEX_POINT ( 'NONE', #113754 ) ;
#116664=CARTESIAN_POINT ( 'NONE',  ( 3.099999999999945022, 12.50000000000000000, -0.3464101615137783474 ) ) ;
#116665=DIRECTION ( 'NONE',  ( 0.000000000000000000, -0.000000000000000000, 1.000000000000000000 ) ) ;
#116666=FACE_OUTER_BOUND ( 'NONE', #122713, .T. ) ;
#116667=DIRECTION ( 'NONE',  ( -0.000000000000000000, -1.000000000000000000, -0.000000000000000000 ) ) ;
#116668=EDGE_LOOP ( 'NONE', ( #68421, #107222 ) ) ;
#116669=EDGE_CURVE ( 'NONE', #82548, #108166, #59440, .T. ) ;
#116670=AXIS2_PLACEMENT_3D ( 'NONE', #73158, #93439, #111797 ) ;
#116671=CARTESIAN_POINT ( 'NONE',  ( -14.59999999999998366, 12.50000000000000000, -1.084202172485504434E-16 ) ) ;
#116672=DIRECTION ( 'NONE',  ( 0.000000000000000000, -0.9999939076577903929, 0.003490651415223739937 ) ) ;
#116673=EDGE_LOOP ( 'NONE', ( #74293, #96219, #31946, #11798 ) ) ;
#116674=DIRECTION ( 'NONE',  ( 0.000000000000000000, 0.000000000000000000, -1.000000000000000000 ) ) ;
#116675=DIRECTION ( 'NONE',  ( -4.274815082592931898E-19, -0.9999939076577903929, -0.003490651415223739937 ) ) ;
#116676=AXIS2_PLACEMENT_3D ( 'NONE', #8344, #97375, #118949 ) ;
#116677=LINE ( 'NONE', #98317, #26122 ) ;
#116678=AXIS2_PLACEMENT_3D ( 'NONE', #43154, #111200, #62777 ) ;
#116679=EDGE_LOOP ( 'NONE', ( #107690, #17768 ) ) ;
#116680=DIRECTION ( 'NONE',  ( -0.000000000000000000, -1.000000000000000000, -0.000000000000000000 ) ) ;
#116681=VERTEX_POINT ( 'NONE', #81696 ) ;
#116682=FACE_OUTER_BOUND ( 'NONE', #44996, .T. ) ;
#116683=LINE ( 'NONE', #125227, #121974 ) ;
#116684=CARTESIAN_POINT ( 'NONE',  ( 7.099999999999926814, 12.50000000000000000, -2.276824562219559311E-15 ) ) ;
#116685=VERTEX_POINT ( 'NONE', #94101 ) ;
#116686=AXIS2_PLACEMENT_3D ( 'NONE', #74562, #123640, #83107 ) ;
#116687=FACE_OUTER_BOUND ( 'NONE', #93149, .T. ) ;
#116688=CARTESIAN_POINT ( 'NONE',  ( 11.84999999999990372, 2.500000000000000000, -6.148780366869526226 ) ) ;
#116689=VERTEX_POINT ( 'NONE', #92161 ) ;
#116690=ORIENTED_EDGE ( 'NONE', *, *, #1946, .F. ) ;
#116691=DIRECTION ( 'NONE',  ( 0.000000000000000000, 1.000000000000000000, 0.000000000000000000 ) ) ;
#116692=AXIS2_PLACEMENT_3D ( 'NONE', #51618, #32644, #81701 ) ;
#116693=ADVANCED_FACE ( 'NONE', ( #13591 ), #28120, .T. ) ;
#116694=EDGE_LOOP ( 'NONE', ( #127665, #939, #66276, #21293 ) ) ;
#116696=DIRECTION ( 'NONE',  ( 0.000000000000000000, 1.000000000000000000, 0.000000000000000000 ) ) ;
#116697=DIRECTION ( 'NONE',  ( 0.000000000000000000, 1.000000000000000000, 0.000000000000000000 ) ) ;
#116698=ORIENTED_EDGE ( 'NONE', *, *, #35573, .T. ) ;
#116699=ORIENTED_EDGE ( 'NONE', *, *, #59793, .T. ) ;
#116700=DIRECTION ( 'NONE',  ( -0.000000000000000000, -1.000000000000000000, -0.000000000000000000 ) ) ;
#116701=LINE ( 'NONE', #25104, #19207 ) ;
#116702=AXIS2_PLACEMENT_3D ( 'NONE', #360, #21302, #51439 ) ;
#116703=VERTEX_POINT ( 'NONE', #43100 ) ;
#116704=EDGE_CURVE ( 'NONE', #93541, #103724, #121616, .T. ) ;
#116705=DIRECTION ( 'NONE',  ( -0.000000000000000000, 1.000000000000000000, -0.000000000000000000 ) ) ;
#116706=DIRECTION ( 'NONE',  ( -0.000000000000000000, -1.000000000000000000, -0.000000000000000000 ) ) ;
#116707=VECTOR ( 'NONE', #89147, 1000.000000000000000 ) ;
#116708=CARTESIAN_POINT ( 'NONE',  ( 8.299999999999922551, 2.500000000000000000, 4.230127018922196669 ) ) ;
#116709=LINE ( 'NONE', #68254, #38371 ) ;
#116710=DIRECTION ( 'NONE',  ( 0.000000000000000000, 0.000000000000000000, 1.000000000000000000 ) ) ;
#116711=CARTESIAN_POINT ( 'NONE',  ( 10.39999999999991509, 12.50000000000000000, -0.6928203230275542523 ) ) ;
#116712=CONICAL_SURFACE ( 'NONE', #60317, 0.1000000000000002554, 0.003490658503988666988 ) ;
#116713=EDGE_LOOP ( 'NONE', ( #112439, #120643 ) ) ;
#116714=ORIENTED_EDGE ( 'NONE', *, *, #112419, .F. ) ;
#116715=ORIENTED_EDGE ( 'NONE', *, *, #116660, .F. ) ;
#116716=ORIENTED_EDGE ( 'NONE', *, *, #17651, .F. ) ;
#116717=DIRECTION ( 'NONE',  ( 0.000000000000000000, 1.000000000000000000, 0.000000000000000000 ) ) ;
#116718=FACE_OUTER_BOUND ( 'NONE', #12164, .T. ) ;
#116719=DIRECTION ( 'NONE',  ( 0.000000000000000000, 0.000000000000000000, 1.000000000000000000 ) ) ;
#116720=AXIS2_PLACEMENT_3D ( 'NONE', #13833, #24312, #81305 ) ;
#116721=EDGE_LOOP ( 'NONE', ( #45449, #48483, #22123, #79325 ) ) ;
#116722=FACE_BOUND ( 'NONE', #99059, .T. ) ;
#116723=LINE ( 'NONE', #79402, #56286 ) ;
#116724=CARTESIAN_POINT ( 'NONE',  ( 8.099999999999923261, 2.500000000000000000, 4.776537180435972196 ) ) ;
#116725=CARTESIAN_POINT ( 'NONE',  ( 7.699999999999925571, 2.500000000000000000, 3.983716857408420076 ) ) ;
#116726=VECTOR ( 'NONE', #89594, 1000.000000000000000 ) ;
#116727=DIRECTION ( 'NONE',  ( -0.000000000000000000, -1.000000000000000000, -0.000000000000000000 ) ) ;
#116728=DIRECTION ( 'NONE',  ( 0.000000000000000000, 0.000000000000000000, 1.000000000000000000 ) ) ;
#116729=CARTESIAN_POINT ( 'NONE',  ( -8.350000000000012079, 12.50000000000000000, 1.472243186433545459 ) ) ;
#116730=CARTESIAN_POINT ( 'NONE',  ( -7.500000000000016875, 2.500000000000000000, 0.6928203230275494784 ) ) ;
#116731=CARTESIAN_POINT ( 'NONE',  ( 9.799999999999918998, 2.500000000000000000, -0.3464101615137782364 ) ) ;
#116732=DIRECTION ( 'NONE',  ( 0.000000000000000000, 0.000000000000000000, 1.000000000000000000 ) ) ;
#116733=CARTESIAN_POINT ( 'NONE',  ( -8.750000000000005329, 2.500000000000000000, 5.902370205355745192 ) ) ;
#116734=EDGE_CURVE ( 'NONE', #120381, #24974, #128400, .T. ) ;
#116735=ORIENTED_EDGE ( 'NONE', *, *, #127155, .T. ) ;
#116736=ORIENTED_EDGE ( 'NONE', *, *, #48690, .T. ) ;
#116737=ORIENTED_EDGE ( 'NONE', *, *, #62871, .F. ) ;
#116738=ORIENTED_EDGE ( 'NONE', *, *, #123069, .F. ) ;
#116739=CARTESIAN_POINT ( 'NONE',  ( 17.49100792770858703, -2.144659849949841490, -4.220823783475863955 ) ) ;
#116740=AXIS2_PLACEMENT_3D ( 'NONE', #39945, #70682, #79851 ) ;
#116741=CARTESIAN_POINT ( 'NONE',  ( 1.249999999999988454, 12.50000000000000000, 2.099970236277060032 ) ) ;
#116742=EDGE_LOOP ( 'NONE', ( #109778, #76957, #107025, #40531 ) ) ;
#116743=VERTEX_POINT ( 'NONE', #31975 ) ;
#116744=ORIENTED_EDGE ( 'NONE', *, *, #118786, .F. ) ;
#116745=DIRECTION ( 'NONE',  ( -0.000000000000000000, -1.000000000000000000, -0.000000000000000000 ) ) ;
#116746=EDGE_CURVE ( 'NONE', #95423, #62529, #63632, .T. ) ;
#116747=AXIS2_PLACEMENT_3D ( 'NONE', #2027, #121803, #42630 ) ;
#116748=CIRCLE ( 'NONE', #45755, 0.1000000000000000472 ) ;
#116749=CARTESIAN_POINT ( 'NONE',  ( 7.314170287673361415, -2.499999999999618083, 9.688393442490539798 ) ) ;
#116750=CIRCLE ( 'NONE', #22689, 0.1000000000000000472 ) ;
#116751=DIRECTION ( 'NONE',  ( -0.000000000000000000, 1.000000000000000000, -0.000000000000000000 ) ) ;
#116752=DIRECTION ( 'NONE',  ( 0.000000000000000000, 0.000000000000000000, 1.000000000000000000 ) ) ;
#116754=EDGE_CURVE ( 'NONE', #79916, #71153, #23921, .T. ) ;
#116755=ADVANCED_FACE ( 'NONE', ( #74464 ), #92879, .T. ) ;
#116756=VERTEX_POINT ( 'NONE', #123545 ) ;
#116757=AXIS2_PLACEMENT_3D ( 'NONE', #10513, #41294, #100824 ) ;
#116758=ORIENTED_EDGE ( 'NONE', *, *, #31680, .F. ) ;
#116759=AXIS2_PLACEMENT_3D ( 'NONE', #57380, #29855, #97304 ) ;
#116760=ORIENTED_EDGE ( 'NONE', *, *, #96978, .F. ) ;
#116761=ORIENTED_EDGE ( 'NONE', *, *, #117499, .T. ) ;
#116762=ADVANCED_FACE ( 'NONE', ( #124208 ), #9246, .T. ) ;
#116763=AXIS2_PLACEMENT_3D ( 'NONE', #11293, #42725, #10627 ) ;
#116764=DIRECTION ( 'NONE',  ( -0.000000000000000000, 1.000000000000000000, -0.000000000000000000 ) ) ;
#116765=ORIENTED_EDGE ( 'NONE', *, *, #122846, .T. ) ;
#116766=EDGE_CURVE ( 'NONE', #24092, #33748, #32254, .T. ) ;
#116767=EDGE_LOOP ( 'NONE', ( #110948, #115495 ) ) ;
#116768=AXIS2_PLACEMENT_3D ( 'NONE', #108324, #67082, #19290 ) ;
#116769=CARTESIAN_POINT ( 'NONE',  ( 2.499999999999948930, 12.50000000000000000, -0.6277270498435166823 ) ) ;
#116770=AXIS2_PLACEMENT_3D ( 'NONE', #37298, #30057, #119072 ) ;
#116771=DIRECTION ( 'NONE',  ( 0.000000000000000000, 0.000000000000000000, -1.000000000000000000 ) ) ;
#116772=DIRECTION ( 'NONE',  ( 0.000000000000000000, 0.000000000000000000, -1.000000000000000000 ) ) ;
#116773=CARTESIAN_POINT ( 'NONE',  ( 11.69999999999990514, 2.500000000000000000, -0.1000000000000022815 ) ) ;
#116774=CARTESIAN_POINT ( 'NONE',  ( 9.799999999999915445, 12.50000000000000000, -4.676537180435977881 ) ) ;
#116775=ORIENTED_EDGE ( 'NONE', *, *, #18192, .F. ) ;
#116776=DIRECTION ( 'NONE',  ( 0.000000000000000000, 0.000000000000000000, -1.000000000000000000 ) ) ;
#116777=ORIENTED_EDGE ( 'NONE', *, *, #30090, .T. ) ;
#116778=FACE_OUTER_BOUND ( 'NONE', #110954, .T. ) ;
#116779=ORIENTED_EDGE ( 'NONE', *, *, #18743, .T. ) ;
#116780=DIRECTION ( 'NONE',  ( 0.000000000000000000, 0.000000000000000000, -1.000000000000000000 ) ) ;
#116781=PLANE ( 'NONE',  #38607 ) ;
#116782=VECTOR ( 'NONE', #49225, 1000.000000000000000 ) ;
#116783=EDGE_LOOP ( 'NONE', ( #68436, #21166 ) ) ;
#116784=DIRECTION ( 'NONE',  ( 0.000000000000000000, 0.000000000000000000, 1.000000000000000000 ) ) ;
#116785=LINE ( 'NONE', #36328, #118810 ) ;
#116786=ORIENTED_EDGE ( 'NONE', *, *, #54256, .T. ) ;
#116787=EDGE_CURVE ( 'NONE', #24257, #24371, #57362, .T. ) ;
#116788=CIRCLE ( 'NONE', #18600, 0.06509327318403745899 ) ;
#116789=CARTESIAN_POINT ( 'NONE',  ( -1.050000000000038236, 2.500000000000000000, -6.148780366869526226 ) ) ;
#116790=VERTEX_POINT ( 'NONE', #17453 ) ;
#116791=ORIENTED_EDGE ( 'NONE', *, *, #58420, .F. ) ;
#116792=CARTESIAN_POINT ( 'NONE',  ( 3.149999999999946176, 2.500000000000000000, -6.148780366869526226 ) ) ;
#116795=CARTESIAN_POINT ( 'NONE',  ( -5.600000000000020073, 12.50000000000000000, 0.2813168883297362810 ) ) ;
#116797=AXIS2_PLACEMENT_3D ( 'NONE', #23197, #33052, #990 ) ;
#116798=EDGE_CURVE ( 'NONE', #80857, #40877, #47589, .T. ) ;
#116799=CIRCLE ( 'NONE', #118867, 0.1000000000000000472 ) ;
#116800=LINE ( 'NONE', #25858, #29051 ) ;
#116801=FACE_OUTER_BOUND ( 'NONE', #49234, .T. ) ;
#116802=EDGE_CURVE ( 'NONE', #55527, #97550, #65268, .T. ) ;
#116803=AXIS2_PLACEMENT_3D ( 'NONE', #55273, #95194, #63805 ) ;
#116804=EDGE_CURVE ( 'NONE', #10727, #249, #5067, .T. ) ;
#116806=ORIENTED_EDGE ( 'NONE', *, *, #33435, .T. ) ;
#116807=DIRECTION ( 'NONE',  ( -4.274815082592931898E-19, -0.9999939076577903929, -0.003490651415223739937 ) ) ;
#116808=ORIENTED_EDGE ( 'NONE', *, *, #73358, .F. ) ;
#116809=CONICAL_SURFACE ( 'NONE', #123088, 0.1000000000000002554, 0.003490658503988666988 ) ;
#116810=CIRCLE ( 'NONE', #62552, 0.1000000000000002554 ) ;
#116811=EDGE_CURVE ( 'NONE', #13161, #117090, #103339, .T. ) ;
#116812=DIRECTION ( 'NONE',  ( -4.274815082592931898E-19, -0.9999939076577903929, -0.003490651415223739937 ) ) ;
#116813=CARTESIAN_POINT ( 'NONE',  ( 14.39999999999989555, 2.500000000000000000, -0.4464101615137782142 ) ) ;
#116814=DIRECTION ( 'NONE',  ( -0.000000000000000000, -1.000000000000000000, -0.000000000000000000 ) ) ;
#116815=LINE ( 'NONE', #127937, #104474 ) ;
#116816=FACE_OUTER_BOUND ( 'NONE', #22465, .T. ) ;
#116818=EDGE_CURVE ( 'NONE', #23967, #86001, #54806, .T. ) ;
#116819=CONICAL_SURFACE ( 'NONE', #106363, 0.1000000000000000472, 0.003490658503988666988 ) ;
#116820=EDGE_CURVE ( 'NONE', #84308, #56285, #46906, .T. ) ;
#116821=FACE_OUTER_BOUND ( 'NONE', #4199, .T. ) ;
#116822=FACE_OUTER_BOUND ( 'NONE', #113941, .T. ) ;
#116823=VERTEX_POINT ( 'NONE', #126790 ) ;
#116824=DIRECTION ( 'NONE',  ( 0.000000000000000000, 0.000000000000000000, 1.000000000000000000 ) ) ;
#116825=VERTEX_POINT ( 'NONE', #7639 ) ;
#116826=VERTEX_POINT ( 'NONE', #45659 ) ;
#116827=DIRECTION ( 'NONE',  ( 0.000000000000000000, 1.000000000000000000, 0.000000000000000000 ) ) ;
#116828=AXIS2_PLACEMENT_3D ( 'NONE', #61851, #82785, #43504 ) ;
#116829=ORIENTED_EDGE ( 'NONE', *, *, #76359, .T. ) ;
#116830=CARTESIAN_POINT ( 'NONE',  ( -6.250000000000019540, 2.500000000000000000, -7.188010851410854052 ) ) ;
#116831=LINE ( 'NONE', #17992, #98714 ) ;
#116832=CARTESIAN_POINT ( 'NONE',  ( 7.499999999999925393, 2.500000000000000000, -0.6928203230275541413 ) ) ;
#116833=VERTEX_POINT ( 'NONE', #15525 ) ;
#116834=FACE_BOUND ( 'NONE', #45396, .T. ) ;
#116835=CIRCLE ( 'NONE', #31191, 0.1000000000000000472 ) ;
#116836=LINE ( 'NONE', #54683, #43215 ) ;
#116837=ORIENTED_EDGE ( 'NONE', *, *, #89471, .F. ) ;
#116838=FACE_OUTER_BOUND ( 'NONE', #45422, .T. ) ;
#116839=CARTESIAN_POINT ( 'NONE',  ( 1.899999999999949507, 12.50000000000000000, 4.676537180435972552 ) ) ;
#116840=VECTOR ( 'NONE', #108279, 1000.000000000000000 ) ;
#116841=ORIENTED_EDGE ( 'NONE', *, *, #52772, .F. ) ;
#116842=AXIS2_PLACEMENT_3D ( 'NONE', #41146, #90866, #81687 ) ;
#116843=AXIS2_PLACEMENT_3D ( 'NONE', #26939, #125142, #76685 ) ;
#116844=EDGE_CURVE ( 'NONE', #52645, #108881, #74088, .T. ) ;
#116845=ORIENTED_EDGE ( 'NONE', *, *, #6534, .F. ) ;
#116846=ORIENTED_EDGE ( 'NONE', *, *, #96226, .T. ) ;
#116847=CARTESIAN_POINT ( 'NONE',  ( 4.799999999999937650, 2.500000000000000000, -0.4464101615137782142 ) ) ;
#116848=DIRECTION ( 'NONE',  ( 0.000000000000000000, 0.000000000000000000, 1.000000000000000000 ) ) ;
#116849=CARTESIAN_POINT ( 'NONE',  ( -3.749999999999991562, 2.500000000000000000, 6.395190528383296602 ) ) ;
#116850=FACE_BOUND ( 'NONE', #68403, .T. ) ;
#116851=EDGE_LOOP ( 'NONE', ( #121185, #75690 ) ) ;
#116852=AXIS2_PLACEMENT_3D ( 'NONE', #117986, #27661, #87231 ) ;
#116855=ADVANCED_FACE ( 'NONE', ( #116944 ), #34399, .T. ) ;
#116856=CIRCLE ( 'NONE', #18582, 0.06509327318403745899 ) ;
#116858=FACE_OUTER_BOUND ( 'NONE', #65561, .T. ) ;
#116859=DIRECTION ( 'NONE',  ( 0.000000000000000000, -0.9999939076577903929, 0.003490651415223739937 ) ) ;
#116860=CARTESIAN_POINT ( 'NONE',  ( 2.699999999999945555, 2.500000000000000000, 3.883716857408420431 ) ) ;
#116861=CARTESIAN_POINT ( 'NONE',  ( -5.800000000000022027, 2.500000000000000000, -4.230127018922201998 ) ) ;
#116862=ORIENTED_EDGE ( 'NONE', *, *, #42754, .T. ) ;
#116863=ORIENTED_EDGE ( 'NONE', *, *, #8599, .T. ) ;
#116864=ORIENTED_EDGE ( 'NONE', *, *, #17479, .T. ) ;
#116865=ORIENTED_EDGE ( 'NONE', *, *, #107150, .F. ) ;
#116866=ORIENTED_EDGE ( 'NONE', *, *, #62877, .T. ) ;
#116867=CONICAL_SURFACE ( 'NONE', #91853, 0.09999999999999982514, 0.003490658503988666988 ) ;
#116868=DIRECTION ( 'NONE',  ( 0.000000000000000000, 0.000000000000000000, 1.000000000000000000 ) ) ;
#116869=CARTESIAN_POINT ( 'NONE',  ( 8.549999999999920774, 12.50000000000000000, 6.148780366869520897 ) ) ;
#116870=EDGE_LOOP ( 'NONE', ( #109971, #43019 ) ) ;
#116871=FACE_BOUND ( 'NONE', #85808, .T. ) ;
#116872=CARTESIAN_POINT ( 'NONE',  ( 7.099999999999928590, 2.500000000000000000, 4.430127018922196847 ) ) ;
#116873=CARTESIAN_POINT ( 'NONE',  ( 12.04999999999990479, 12.50000000000000000, -6.495190528383302464 ) ) ;
#116874=FACE_OUTER_BOUND ( 'NONE', #125627, .T. ) ;
#116875=PLANE ( 'NONE',  #103380 ) ;
#116876=FACE_OUTER_BOUND ( 'NONE', #49991, .T. ) ;
#116877=EDGE_LOOP ( 'NONE', ( #13603, #94982, #65322, #71862 ) ) ;
#116878=CONICAL_SURFACE ( 'NONE', #20757, 0.09999999999999982514, 0.003490658503988666988 ) ;
#116879=DIRECTION ( 'NONE',  ( 0.000000000000000000, 1.000000000000000000, 0.000000000000000000 ) ) ;
#116880=CONICAL_SURFACE ( 'NONE', #60493, 0.09999999999999982514, 0.003490658503988666988 ) ;
#116881=ORIENTED_EDGE ( 'NONE', *, *, #80383, .F. ) ;
#116882=EDGE_LOOP ( 'NONE', ( #3396, #23972 ) ) ;
#116883=ORIENTED_EDGE ( 'NONE', *, *, #60199, .T. ) ;
#116884=CARTESIAN_POINT ( 'NONE',  ( 9.349999999999919709, 12.50000000000000000, -6.906693963081115939 ) ) ;
#116885=CARTESIAN_POINT ( 'NONE',  ( 14.18215599311778696, 2.499999999999998224, 6.639800458426438290 ) ) ;
#116886=DIRECTION ( 'NONE',  ( -0.000000000000000000, -1.000000000000000000, -0.000000000000000000 ) ) ;
#116887=AXIS2_PLACEMENT_3D ( 'NONE', #127868, #97766, #125923 ) ;
#116888=EDGE_LOOP ( 'NONE', ( #30553, #68345 ) ) ;
#116889=CARTESIAN_POINT ( 'NONE',  ( 7.173569985890439149, 2.499999999999999556, -8.713264184206867213 ) ) ;
#116890=EDGE_CURVE ( 'NONE', #64922, #65156, #75738, .T. ) ;
#116891=DIRECTION ( 'NONE',  ( 0.000000000000000000, 0.000000000000000000, -1.000000000000000000 ) ) ;
#116892=AXIS2_PLACEMENT_3D ( 'NONE', #1705, #101213, #100555 ) ;
#116893=DIRECTION ( 'NONE',  ( 0.000000000000000000, 0.000000000000000000, 1.000000000000000000 ) ) ;
#116894=AXIS2_PLACEMENT_3D ( 'NONE', #43639, #92725, #62632 ) ;
#116896=DIRECTION ( 'NONE',  ( -0.000000000000000000, 1.000000000000000000, -0.000000000000000000 ) ) ;
#116897=DIRECTION ( 'NONE',  ( 0.000000000000000000, 0.000000000000000000, 1.000000000000000000 ) ) ;
#116898=AXIS2_PLACEMENT_3D ( 'NONE', #94506, #42206, #122691 ) ;
#116899=EDGE_CURVE ( 'NONE', #89926, #119243, #107127, .T. ) ;
#116900=LINE ( 'NONE', #16757, #3520 ) ;
#116901=EDGE_CURVE ( 'NONE', #1265, #79987, #115660, .T. ) ;
#116902=EDGE_LOOP ( 'NONE', ( #21219, #30195 ) ) ;
#116903=DIRECTION ( 'NONE',  ( 0.000000000000000000, 0.000000000000000000, -1.000000000000000000 ) ) ;
#116904=CIRCLE ( 'NONE', #75066, 0.09999999999999982514 ) ;
#116905=AXIS2_PLACEMENT_3D ( 'NONE', #122804, #23296, #44228 ) ;
#116906=ORIENTED_EDGE ( 'NONE', *, *, #108916, .F. ) ;
#116907=ORIENTED_EDGE ( 'NONE', *, *, #52680, .T. ) ;
#116908=DIRECTION ( 'NONE',  ( 0.000000000000000000, 0.000000000000000000, -1.000000000000000000 ) ) ;
#116909=EDGE_CURVE ( 'NONE', #112155, #43428, #26016, .T. ) ;
#116910=EDGE_CURVE ( 'NONE', #42980, #11927, #90806, .T. ) ;
#116912=CARTESIAN_POINT ( 'NONE',  ( -7.500000000000015099, 2.500000000000000000, -5.022947341949754119 ) ) ;
#116913=ADVANCED_FACE ( 'NONE', ( #105857 ), #35198, .T. ) ;
#116914=EDGE_LOOP ( 'NONE', ( #96945, #116337 ) ) ;
#116915=ORIENTED_EDGE ( 'NONE', *, *, #55205, .F. ) ;
#116916=DIRECTION ( 'NONE',  ( -0.000000000000000000, 1.000000000000000000, -0.000000000000000000 ) ) ;
#116917=CARTESIAN_POINT ( 'NONE',  ( 10.79999999999991012, 2.500000000000000000, -4.430127018922202176 ) ) ;
#116918=DIRECTION ( 'NONE',  ( 0.000000000000000000, 0.000000000000000000, 1.000000000000000000 ) ) ;
#116919=VERTEX_POINT ( 'NONE', #25343 ) ;
#116920=ORIENTED_EDGE ( 'NONE', *, *, #13337, .T. ) ;
#116921=DIRECTION ( 'NONE',  ( 0.000000000000000000, 0.000000000000000000, 1.000000000000000000 ) ) ;
#116922=EDGE_LOOP ( 'NONE', ( #64355, #48613 ) ) ;
#116923=CARTESIAN_POINT ( 'NONE',  ( 13.54999999999989946, 2.500000000000000000, 2.611473670974873151 ) ) ;
#116924=CIRCLE ( 'NONE', #129585, 0.06509327318403745899 ) ;
#116925=DIRECTION ( 'NONE',  ( -0.000000000000000000, -1.000000000000000000, -0.000000000000000000 ) ) ;
#116926=VERTEX_POINT ( 'NONE', #46953 ) ;
#116927=DIRECTION ( 'NONE',  ( -0.000000000000000000, -1.000000000000000000, -0.000000000000000000 ) ) ;
#116928=CARTESIAN_POINT ( 'NONE',  ( -13.54999999999998828, 12.50000000000000000, 1.818653347947325472 ) ) ;
#116929=FACE_OUTER_BOUND ( 'NONE', #127120, .T. ) ;
#116930=CARTESIAN_POINT ( 'NONE',  ( -11.64999999999999680, 12.50000000000000000, -6.495190528383298911 ) ) ;
#116931=CONICAL_SURFACE ( 'NONE', #85553, 0.1000000000000002554, 0.003490658503988666988 ) ;
#116932=ORIENTED_EDGE ( 'NONE', *, *, #80606, .T. ) ;
#116933=AXIS2_PLACEMENT_3D ( 'NONE', #121449, #91352, #29232 ) ;
#116934=AXIS2_PLACEMENT_3D ( 'NONE', #62840, #13721, #31456 ) ;
#116935=CARTESIAN_POINT ( 'NONE',  ( -11.89999999999999680, 12.50000000000000000, -4.611443907251937979 ) ) ;
#116936=FACE_OUTER_BOUND ( 'NONE', #67089, .T. ) ;
#116937=ORIENTED_EDGE ( 'NONE', *, *, #109597, .F. ) ;
#116938=EDGE_LOOP ( 'NONE', ( #110811, #107619, #4477, #12956 ) ) ;
#116940=CARTESIAN_POINT ( 'NONE',  ( -3.350000000000028511, 2.500000000000000000, 2.857883832488649301 ) ) ;
#116941=CARTESIAN_POINT ( 'NONE',  ( -14.54999999999998472, 2.500000000000000000, -2.265063509461099578 ) ) ;
#116942=DIRECTION ( 'NONE',  ( 0.000000000000000000, 1.000000000000000000, 0.000000000000000000 ) ) ;
#116943=CONICAL_SURFACE ( 'NONE', #6214, 0.1000000000000002554, 0.003490658503988666988 ) ;
#116944=FACE_OUTER_BOUND ( 'NONE', #98, .T. ) ;
#116945=DIRECTION ( 'NONE',  ( 0.000000000000000000, 0.000000000000000000, 1.000000000000000000 ) ) ;
#116946=CONICAL_SURFACE ( 'NONE', #37557, 0.09999999999999982514, 0.003490658503988666988 ) ;
#116947=CIRCLE ( 'NONE', #20828, 0.06509327318403745899 ) ;
#116948=LINE ( 'NONE', #16160, #25880 ) ;
#116949=DIRECTION ( 'NONE',  ( -0.000000000000000000, 1.000000000000000000, -0.000000000000000000 ) ) ;
#116950=CARTESIAN_POINT ( 'NONE',  ( 8.349999999999923261, 2.500000000000000000, 1.372243186433545370 ) ) ;
#116951=EDGE_CURVE ( 'NONE', #81732, #97929, #59544, .T. ) ;
#116952=ADVANCED_FACE ( 'NONE', ( #26657 ), #6980, .T. ) ;
#116953=EDGE_CURVE ( 'NONE', #16115, #74932, #124358, .T. ) ;
#116954=DIRECTION ( 'NONE',  ( -0.000000000000000000, -1.000000000000000000, -0.000000000000000000 ) ) ;
#116955=EDGE_LOOP ( 'NONE', ( #122565, #36914 ) ) ;
#116956=ADVANCED_FACE ( 'NONE', ( #117575 ), #36541, .T. ) ;
#116957=AXIS2_PLACEMENT_3D ( 'NONE', #119987, #30334, #108858 ) ;
#116958=FACE_OUTER_BOUND ( 'NONE', #12120, .T. ) ;
#116959=EDGE_CURVE ( 'NONE', #81870, #21966, #61670, .T. ) ;
#116961=DIRECTION ( 'NONE',  ( 0.000000000000000000, 0.000000000000000000, -1.000000000000000000 ) ) ;
#116962=DIRECTION ( 'NONE',  ( 0.000000000000000000, 0.000000000000000000, 1.000000000000000000 ) ) ;
#116963=VERTEX_POINT ( 'NONE', #109050 ) ;
#116964=ADVANCED_FACE ( 'NONE', ( #99909 ), #99230, .T. ) ;
#116965=DIRECTION ( 'NONE',  ( 0.000000000000000000, -0.9999939076577903929, 0.003490651415223739937 ) ) ;
#116966=EDGE_CURVE ( 'NONE', #67328, #48532, #82510, .T. ) ;
#116967=DIRECTION ( 'NONE',  ( 0.000000000000000000, 0.000000000000000000, -1.000000000000000000 ) ) ;
#116968=FACE_OUTER_BOUND ( 'NONE', #10230, .T. ) ;
#116970=EDGE_CURVE ( 'NONE', #92073, #3679, #50808, .T. ) ;
#116971=ORIENTED_EDGE ( 'NONE', *, *, #110713, .T. ) ;
#116972=EDGE_LOOP ( 'NONE', ( #82232, #103194 ) ) ;
#116973=ORIENTED_EDGE ( 'NONE', *, *, #29898, .T. ) ;
#116974=ORIENTED_EDGE ( 'NONE', *, *, #3858, .F. ) ;
#116975=PLANE ( 'NONE',  #98846 ) ;
#116976=AXIS2_PLACEMENT_3D ( 'NONE', #25469, #65401, #105340 ) ;
#116977=PLANE ( 'NONE',  #128043 ) ;
#116978=LINE ( 'NONE', #60036, #77605 ) ;
#116979=CARTESIAN_POINT ( 'NONE',  ( 4.399999999999940847, 12.50000000000000000, -3.983716857408426293 ) ) ;
#116980=ORIENTED_EDGE ( 'NONE', *, *, #61409, .T. ) ;
#116981=VECTOR ( 'NONE', #72404, 1000.000000000000000 ) ;
#116982=AXIS2_PLACEMENT_3D ( 'NONE', #37675, #107697, #85473 ) ;
#116983=PLANE ( 'NONE',  #87958 ) ;
#116984=EDGE_LOOP ( 'NONE', ( #57583, #26502, #23764, #79062 ) ) ;
#116985=CARTESIAN_POINT ( 'NONE',  ( 65.40763333645755040, -3.109051995142349867, -5.794606894451852064 ) ) ;
#116986=CARTESIAN_POINT ( 'NONE',  ( 13.80955901302179534, -2.500000000000000000, -7.955427456727499624 ) ) ;
#116987=CARTESIAN_POINT ( 'NONE',  ( 6.249999999999934275, 2.500000000000000000, -7.288010851410854585 ) ) ;
#116988=FACE_OUTER_BOUND ( 'NONE', #114088, .T. ) ;
#116989=ORIENTED_EDGE ( 'NONE', *, *, #115744, .F. ) ;
#116990=CONICAL_SURFACE ( 'NONE', #100293, 0.09999999999999982514, 0.003490658503988666988 ) ;
#116991=AXIS2_PLACEMENT_3D ( 'NONE', #114900, #107004, #127323 ) ;
#116992=ORIENTED_EDGE ( 'NONE', *, *, #112839, .T. ) ;
#116993=ORIENTED_EDGE ( 'NONE', *, *, #4191, .F. ) ;
#116994=ORIENTED_EDGE ( 'NONE', *, *, #73186, .T. ) ;
#116995=CARTESIAN_POINT ( 'NONE',  ( -11.44999999999999929, 12.50000000000000000, -6.148780366869522673 ) ) ;
#116996=CARTESIAN_POINT ( 'NONE',  ( -7.300000000000018474, 2.500000000000000000, -4.083716857408426826 ) ) ;
#116997=PLANE ( 'NONE',  #25285 ) ;
#116998=FACE_BOUND ( 'NONE', #52326, .T. ) ;
#116999=DIRECTION ( 'NONE',  ( 0.000000000000000000, 0.000000000000000000, -1.000000000000000000 ) ) ;
#117000=DIRECTION ( 'NONE',  ( 0.000000000000000000, 1.000000000000000000, 0.000000000000000000 ) ) ;
#117001=CARTESIAN_POINT ( 'NONE',  ( -7.300000000000013145, 12.50000000000000000, 3.918623584224382839 ) ) ;
#117002=DIRECTION ( 'NONE',  ( -0.000000000000000000, 1.000000000000000000, -0.000000000000000000 ) ) ;
#117003=EDGE_CURVE ( 'NONE', #13612, #51768, #21970, .T. ) ;
#117005=DIRECTION ( 'NONE',  ( 0.000000000000000000, 1.000000000000000000, 0.000000000000000000 ) ) ;
#117006=CARTESIAN_POINT ( 'NONE',  ( -4.550000000000022915, 12.50000000000000000, 2.165063509461097713 ) ) ;
#117007=AXIS2_PLACEMENT_3D ( 'NONE', #62438, #13307, #114101 ) ;
#117008=CIRCLE ( 'NONE', #94053, 0.1000000000000002554 ) ;
#117009=CARTESIAN_POINT ( 'NONE',  ( 0.8499999999999545697, 2.500000000000000000, -1.472243186433550122 ) ) ;
#117010=VERTEX_POINT ( 'NONE', #107789 ) ;
#117011=ORIENTED_EDGE ( 'NONE', *, *, #83984, .F. ) ;
#117012=ORIENTED_EDGE ( 'NONE', *, *, #24178, .T. ) ;
#117013=ORIENTED_EDGE ( 'NONE', *, *, #17448, .F. ) ;
#117014=DIRECTION ( 'NONE',  ( -0.000000000000000000, 1.000000000000000000, -0.000000000000000000 ) ) ;
#117015=FACE_BOUND ( 'NONE', #105162, .T. ) ;
#117016=DIRECTION ( 'NONE',  ( 0.000000000000000000, 0.000000000000000000, 1.000000000000000000 ) ) ;
#117017=AXIS2_PLACEMENT_3D ( 'NONE', #46569, #5993, #47240 ) ;
#117018=CARTESIAN_POINT ( 'NONE',  ( -5.850000000000018296, 12.50000000000000000, 7.188010851410848723 ) ) ;
#117019=EDGE_LOOP ( 'NONE', ( #96155, #80963 ) ) ;
#117020=CARTESIAN_POINT ( 'NONE',  ( -7.499999999999980460, 2.500000000000000000, -0.1000000000000022815 ) ) ;
#117021=CARTESIAN_POINT ( 'NONE',  ( -7.900000000000014566, 2.500000000000000000, -3.737306695894649700 ) ) ;
#117022=DIRECTION ( 'NONE',  ( -0.000000000000000000, 1.000000000000000000, -0.000000000000000000 ) ) ;
#117023=VECTOR ( 'NONE', #79065, 1000.000000000000000 ) ;
#117024=VERTEX_POINT ( 'NONE', #68500 ) ;
#117025=CARTESIAN_POINT ( 'NONE',  ( 10.64999999999990976, 12.50000000000000000, -6.213873640053564351 ) ) ;
#117026=DIRECTION ( 'NONE',  ( 0.000000000000000000, 1.000000000000000000, 0.000000000000000000 ) ) ;
#117027=CIRCLE ( 'NONE', #121262, 0.1000000000000002554 ) ;
#117028=CONICAL_SURFACE ( 'NONE', #39728, 0.1000000000000000472, 0.003490658503988666988 ) ;
#117029=ORIENTED_EDGE ( 'NONE', *, *, #2770, .T. ) ;
#117030=CARTESIAN_POINT ( 'NONE',  ( 8.549999999999918998, 2.500000000000000000, -1.818653347947326138 ) ) ;
#117031=CARTESIAN_POINT ( 'NONE',  ( -6.450000000000017941, 2.500000000000000000, -6.941600689897077459 ) ) ;
#117032=CIRCLE ( 'NONE', #20917, 0.06509327318403745899 ) ;
#117033=AXIS2_PLACEMENT_3D ( 'NONE', #113296, #32828, #102820 ) ;
#117034=ORIENTED_EDGE ( 'NONE', *, *, #31751, .T. ) ;
#117035=ADVANCED_FACE ( 'NONE', ( #59356 ), #40752, .T. ) ;
#117036=DIRECTION ( 'NONE',  ( 0.000000000000000000, 0.000000000000000000, 1.000000000000000000 ) ) ;
#117037=CARTESIAN_POINT ( 'NONE',  ( 11.84999999999990727, 2.500000000000000000, 6.841600689897072485 ) ) ;
#117038=EDGE_LOOP ( 'NONE', ( #18912, #22417, #540, #93854 ) ) ;
#117039=CARTESIAN_POINT ( 'NONE',  ( 9.999999999999911182, 2.500000000000000000, -3.637306695894650055 ) ) ;
#117040=AXIS2_PLACEMENT_3D ( 'NONE', #104151, #14457, #54397 ) ;
#117041=ORIENTED_EDGE ( 'NONE', *, *, #91159, .T. ) ;
#117042=ORIENTED_EDGE ( 'NONE', *, *, #2929, .T. ) ;
#117043=EDGE_CURVE ( 'NONE', #123305, #87698, #80270, .T. ) ;
#117044=DIRECTION ( 'NONE',  ( 0.000000000000000000, 0.000000000000000000, 1.000000000000000000 ) ) ;
#117045=EDGE_CURVE ( 'NONE', #6029, #63031, #109693, .T. ) ;
#117046=ORIENTED_EDGE ( 'NONE', *, *, #24281, .T. ) ;
#117047=DIRECTION ( 'NONE',  ( -0.000000000000000000, -1.000000000000000000, -0.000000000000000000 ) ) ;
#117048=FACE_BOUND ( 'NONE', #96898, .T. ) ;
#117049=ORIENTED_EDGE ( 'NONE', *, *, #100405, .T. ) ;
#117050=CARTESIAN_POINT ( 'NONE',  ( 12.09999999999990195, 2.500000000000000000, -0.6928203230275541413 ) ) ;
#117051=VERTEX_POINT ( 'NONE', #10237 ) ;
#117053=CARTESIAN_POINT ( 'NONE',  ( -4.150000000000027889, 12.50000000000000000, -6.560283801567339701 ) ) ;
#117054=EDGE_CURVE ( 'NONE', #92955, #120893, #70445, .T. ) ;
#117055=EDGE_CURVE ( 'NONE', #64042, #75618, #122211, .T. ) ;
#117056=( BOUNDED_CURVE ( )  B_SPLINE_CURVE ( 2, ( #27480, #37967, #17673 ),
 .UNSPECIFIED., .F., .F. ) 
 B_SPLINE_CURVE_WITH_KNOTS ( ( 3, 3 ),
 ( 0.0008083180696985040568, 0.0008883710667521964310 ),
 .UNSPECIFIED. ) 
 CURVE ( )  GEOMETRIC_REPRESENTATION_ITEM ( )  RATIONAL_B_SPLINE_CURVE ( ( 0.9944676636817101345, 0.9972072019273799937, 1.000000000000000000 ) ) 
 REPRESENTATION_ITEM ( '' )  );
#117057=DIRECTION ( 'NONE',  ( 0.000000000000000000, -0.9999939076577903929, 0.003490651415223739937 ) ) ;
#117058=EDGE_CURVE ( 'NONE', #91328, #58594, #42818, .T. ) ;
#117059=DIRECTION ( 'NONE',  ( 0.000000000000000000, 1.000000000000000000, 0.000000000000000000 ) ) ;
#117060=ADVANCED_FACE ( 'NONE', ( #90726 ), #84644, .T. ) ;
#117061=ADVANCED_FACE ( 'NONE', ( #60004 ), #51205, .T. ) ;
#117062=DIRECTION ( 'NONE',  ( -0.000000000000000000, -1.000000000000000000, -0.000000000000000000 ) ) ;
#117063=EDGE_LOOP ( 'NONE', ( #26196, #82800 ) ) ;
#117064=ORIENTED_EDGE ( 'NONE', *, *, #127728, .F. ) ;
#117065=DIRECTION ( 'NONE',  ( -0.000000000000000000, 1.000000000000000000, -0.000000000000000000 ) ) ;
#117066=CARTESIAN_POINT ( 'NONE',  ( 17.37282530749025966, -0.4689596142739139717, 5.357821376857582862 ) ) ;
#117067=AXIS2_PLACEMENT_3D ( 'NONE', #121439, #82830, #51442 ) ;
#117068=LINE ( 'NONE', #96152, #112895 ) ;
#117069=ORIENTED_EDGE ( 'NONE', *, *, #74399, .T. ) ;
#117070=VERTEX_POINT ( 'NONE', #48886 ) ;
#117071=EDGE_LOOP ( 'NONE', ( #43346, #7751, #32648, #78399, #127358, #123350, #58593, #75597, #112912, #100386, #40983, #44841 ) ) ;
#117072=EDGE_CURVE ( 'NONE', #56826, #85037, #98589, .T. ) ;
#117073=CARTESIAN_POINT ( 'NONE',  ( 8.949999999999917577, 2.500000000000000000, -2.511473670974877948 ) ) ;
#117074=CARTESIAN_POINT ( 'NONE',  ( -8.300000000000011369, 12.50000000000000000, -4.395220292106239768 ) ) ;
#117075=EDGE_CURVE ( 'NONE', #104178, #67710, #95024, .T. ) ;
#117076=CARTESIAN_POINT ( 'NONE',  ( 7.899999999999924860, 12.50000000000000000, -4.957854068765716882 ) ) ;
#117078=CONICAL_SURFACE ( 'NONE', #106, 0.1000000000000000472, 0.003490658503988666988 ) ;
#117079=AXIS2_PLACEMENT_3D ( 'NONE', #53298, #44100, #4804 ) ;
#117080=LINE ( 'NONE', #86990, #108006 ) ;
#117081=FACE_OUTER_BOUND ( 'NONE', #13018, .T. ) ;
#117082=CARTESIAN_POINT ( 'NONE',  ( -6.650000000000018119, 2.500000000000000000, -2.957883832488653830 ) ) ;
#117083=FACE_OUTER_BOUND ( 'NONE', #48134, .T. ) ;
#117084=CARTESIAN_POINT ( 'NONE',  ( -11.25000000000000000, 2.500000000000000000, 7.188010851410848723 ) ) ;
#117085=LINE ( 'NONE', #56243, #6033 ) ;
#117086=VERTEX_POINT ( 'NONE', #58691 ) ;
#117087=AXIS2_PLACEMENT_3D ( 'NONE', #72868, #112798, #23117 ) ;
#117088=ORIENTED_EDGE ( 'NONE', *, *, #27418, .T. ) ;
#117089=CARTESIAN_POINT ( 'NONE',  ( 11.69999999999990870, 12.50000000000000000, 4.330127018922196314 ) ) ;
#117090=VERTEX_POINT ( 'NONE', #8924 ) ;
#117091=VERTEX_POINT ( 'NONE', #128747 ) ;
#117092=FACE_OUTER_BOUND ( 'NONE', #2315, .T. ) ;
#117093=CARTESIAN_POINT ( 'NONE',  ( 4.549999999999937650, 2.500000000000000000, 2.065063509461097624 ) ) ;
#117094=CARTESIAN_POINT ( 'NONE',  ( -4.251297162942325111E-14, 2.500000000000000000, -3.737306695894649700 ) ) ;
#117095=FACE_OUTER_BOUND ( 'NONE', #69548, .T. ) ;
#117096=DIRECTION ( 'NONE',  ( 0.000000000000000000, 1.000000000000000000, 0.000000000000000000 ) ) ;
#117097=CARTESIAN_POINT ( 'NONE',  ( -7.300000000000018474, 2.500000000000000000, -4.083716857408426826 ) ) ;
#117098=DIRECTION ( 'NONE',  ( 0.000000000000000000, 0.000000000000000000, 1.000000000000000000 ) ) ;
#117099=EDGE_LOOP ( 'NONE', ( #114981, #66223, #105178, #46183 ) ) ;
#117100=DIRECTION ( 'NONE',  ( 0.000000000000000000, -0.000000000000000000, 1.000000000000000000 ) ) ;
#117101=EDGE_CURVE ( 'NONE', #15129, #63981, #103776, .T. ) ;
#117102=ADVANCED_FACE ( 'NONE', ( #91368 ), #53260, .T. ) ;
#117103=CARTESIAN_POINT ( 'NONE',  ( 9.149999999999916866, 2.500000000000000000, -1.472243186433550122 ) ) ;
#117104=ORIENTED_EDGE ( 'NONE', *, *, #43823, .F. ) ;
#117105=EDGE_CURVE ( 'NONE', #94293, #83874, #14078, .T. ) ;
#117107=EDGE_LOOP ( 'NONE', ( #105169, #10499, #9695, #108062 ) ) ;
#117108=EDGE_CURVE ( 'NONE', #37252, #59946, #88757, .T. ) ;
#117109=ORIENTED_EDGE ( 'NONE', *, *, #17314, .F. ) ;
#117110=CARTESIAN_POINT ( 'NONE',  ( 1.849999999999950573, 2.500000000000000000, -1.818653347947326138 ) ) ;
#117111=FACE_OUTER_BOUND ( 'NONE', #18855, .T. ) ;
#117112=AXIS2_PLACEMENT_3D ( 'NONE', #101395, #121026, #78042 ) ;
#117113=ADVANCED_FACE ( 'NONE', ( #33118 ), #76242, .T. ) ;
#117114=EDGE_LOOP ( 'NONE', ( #101929, #67615 ) ) ;
#117115=CARTESIAN_POINT ( 'NONE',  ( 12.89999999999990266, 2.500000000000000000, 5.022947341949748790 ) ) ;
#117116=DIRECTION ( 'NONE',  ( -0.000000000000000000, 1.000000000000000000, -0.000000000000000000 ) ) ;
#117117=ADVANCED_FACE ( 'NONE', ( #31183 ), #61276, .T. ) ;
#117118=DIRECTION ( 'NONE',  ( -0.000000000000000000, -1.000000000000000000, -0.000000000000000000 ) ) ;
#117120=DIRECTION ( 'NONE',  ( 0.000000000000000000, 0.000000000000000000, 1.000000000000000000 ) ) ;
#117121=EDGE_CURVE ( 'NONE', #128031, #29713, #32354, .T. ) ;
#117122=DIRECTION ( 'NONE',  ( 0.000000000000000000, -0.9999939076577903929, 0.003490651415223739937 ) ) ;
#117123=CIRCLE ( 'NONE', #125458, 0.06509327318403745899 ) ;
#117124=EDGE_LOOP ( 'NONE', ( #29312, #2665 ) ) ;
#117125=CIRCLE ( 'NONE', #115070, 0.06509327318403745899 ) ;
#117126=ORIENTED_EDGE ( 'NONE', *, *, #10963, .T. ) ;
#117127=ORIENTED_EDGE ( 'NONE', *, *, #118125, .T. ) ;
#117128=DIRECTION ( 'NONE',  ( -0.000000000000000000, -1.000000000000000000, -0.000000000000000000 ) ) ;
#117129=AXIS2_PLACEMENT_3D ( 'NONE', #12370, #122982, #123603 ) ;
#117130=CARTESIAN_POINT ( 'NONE',  ( -8.350000000000012079, 12.50000000000000000, -1.472243186433550122 ) ) ;
#117131=AXIS2_PLACEMENT_3D ( 'NONE', #122363, #92231, #90286 ) ;
#117132=ORIENTED_EDGE ( 'NONE', *, *, #118387, .T. ) ;
#117133=CARTESIAN_POINT ( 'NONE',  ( 4.799999999999935874, 12.50000000000000000, 0.3464101615137735735 ) ) ;
#117134=DIRECTION ( 'NONE',  ( 0.000000000000000000, 1.000000000000000000, 0.000000000000000000 ) ) ;
#117135=CARTESIAN_POINT ( 'NONE',  ( 2.499999999999983569, 2.500000000000000000, -4.330127018922201643 ) ) ;
#117136=CARTESIAN_POINT ( 'NONE',  ( 6.249999999999968914, 12.50000000000000000, -6.430097255199264339 ) ) ;
#117137=EDGE_CURVE ( 'NONE', #28419, #47021, #73020, .T. ) ;
#117138=ORIENTED_EDGE ( 'NONE', *, *, #66515, .F. ) ;
#117139=DIRECTION ( 'NONE',  ( 0.000000000000000000, 0.000000000000000000, 1.000000000000000000 ) ) ;
#117140=ORIENTED_EDGE ( 'NONE', *, *, #86344, .F. ) ;
#117141=ORIENTED_EDGE ( 'NONE', *, *, #37332, .T. ) ;
#117142=FACE_OUTER_BOUND ( 'NONE', #19849, .T. ) ;
#117143=VERTEX_POINT ( 'NONE', #11519 ) ;
#117144=CARTESIAN_POINT ( 'NONE',  ( -10.85000000000000142, 12.50000000000000000, -2.857883832488649745 ) ) ;
#117145=FACE_BOUND ( 'NONE', #111597, .T. ) ;
#117146=CARTESIAN_POINT ( 'NONE',  ( 8.349999999999919709, 2.500000000000000000, 5.902370205355745192 ) ) ;
#117147=DIRECTION ( 'NONE',  ( 0.000000000000000000, 1.000000000000000000, 0.000000000000000000 ) ) ;
#117148=CARTESIAN_POINT ( 'NONE',  ( 9.549999999999918998, 2.500000000000000000, -6.495190528383302464 ) ) ;
#117149=EDGE_CURVE ( 'NONE', #95427, #23570, #51463, .T. ) ;
#117150=AXIS2_PLACEMENT_3D ( 'NONE', #128050, #48862, #79596 ) ;
#117151=EDGE_LOOP ( 'NONE', ( #120895, #23659 ) ) ;
#117152=CARTESIAN_POINT ( 'NONE',  ( 1.049999999999954525, 12.50000000000000000, -2.511473670974877948 ) ) ;
#117153=CONICAL_SURFACE ( 'NONE', #52428, 0.1000000000000000472, 0.003490658503988666988 ) ;
#117154=CARTESIAN_POINT ( 'NONE',  ( -0.6000000000000383915, 12.50000000000000000, -3.983716857408426293 ) ) ;
#117155=DIRECTION ( 'NONE',  ( 0.000000000000000000, -0.9999939076577903929, 0.003490651415223739937 ) ) ;
#117156=CARTESIAN_POINT ( 'NONE',  ( 3.349999999999944578, 2.500000000000000000, -5.802370205355749988 ) ) ;
#117157=VERTEX_POINT ( 'NONE', #1687 ) ;
#117158=DIRECTION ( 'NONE',  ( -0.000000000000000000, 1.000000000000000000, -0.000000000000000000 ) ) ;
#117160=CARTESIAN_POINT ( 'NONE',  ( 2.299999999999947864, 2.500000000000000000, 3.983716857408420964 ) ) ;
#117161=VERTEX_POINT ( 'NONE', #41012 ) ;
#117162=DIRECTION ( 'NONE',  ( 0.000000000000000000, 0.000000000000000000, 1.000000000000000000 ) ) ;
#117163=EDGE_CURVE ( 'NONE', #108547, #71302, #74182, .T. ) ;
#117164=DIRECTION ( 'NONE',  ( 0.000000000000000000, 0.000000000000000000, 1.000000000000000000 ) ) ;
#117165=FACE_BOUND ( 'NONE', #1440, .T. ) ;
#117166=DIRECTION ( 'NONE',  ( 0.000000000000000000, 0.000000000000000000, -1.000000000000000000 ) ) ;
#117167=VERTEX_POINT ( 'NONE', #112307 ) ;
#117168=CARTESIAN_POINT ( 'NONE',  ( 13.34999999999990017, 2.500000000000000000, 2.857883832488649301 ) ) ;
#117169=EDGE_LOOP ( 'NONE', ( #31786, #54693 ) ) ;
#117170=EDGE_LOOP ( 'NONE', ( #8129, #14248, #10633, #115856 ) ) ;
#117171=CARTESIAN_POINT ( 'NONE',  ( 16.70850060796086822, 0.4765610498145367302, -5.930927070179643934 ) ) ;
#117173=VERTEX_POINT ( 'NONE', #22648 ) ;
#117175=FACE_OUTER_BOUND ( 'NONE', #58228, .T. ) ;
#117176=FACE_OUTER_BOUND ( 'NONE', #36510, .T. ) ;
#117179=EDGE_CURVE ( 'NONE', #114690, #10201, #103427, .T. ) ;
#117180=CARTESIAN_POINT ( 'NONE',  ( 12.04999999999990479, 12.50000000000000000, 2.165063509461097713 ) ) ;
#117181=CARTESIAN_POINT ( 'NONE',  ( 7.699999999999923794, 2.500000000000000000, -0.2464101615137783419 ) ) ;
#117182=CARTESIAN_POINT ( 'NONE',  ( 7.299999999999926104, 2.500000000000000000, -0.4464101615137782142 ) ) ;
#117183=CARTESIAN_POINT ( 'NONE',  ( 18.46077493896295607, -0.2575262203714185349, -4.048716073870159526 ) ) ;
#117184=ORIENTED_EDGE ( 'NONE', *, *, #6504, .F. ) ;
#117185=CARTESIAN_POINT ( 'NONE',  ( 3.099999999999945466, 2.500000000000000000, 0.4464101615137735513 ) ) ;
#117186=ORIENTED_EDGE ( 'NONE', *, *, #103651, .F. ) ;
#117187=DIRECTION ( 'NONE',  ( -0.000000000000000000, -1.000000000000000000, -0.000000000000000000 ) ) ;
#117188=DIRECTION ( 'NONE',  ( 0.000000000000000000, 0.000000000000000000, 1.000000000000000000 ) ) ;
#117189=AXIS2_PLACEMENT_3D ( 'NONE', #35087, #114267, #44900 ) ;
#117190=ORIENTED_EDGE ( 'NONE', *, *, #64167, .F. ) ;
#117191=DIRECTION ( 'NONE',  ( 0.000000000000000000, -0.9999939076577903929, 0.003490651415223739937 ) ) ;
#117192=ADVANCED_FACE ( 'NONE', ( #112946 ), #80449, .T. ) ;
#117193=DIRECTION ( 'NONE',  ( 0.000000000000000000, 0.000000000000000000, -1.000000000000000000 ) ) ;
#117194=DIRECTION ( 'NONE',  ( 0.000000000000000000, 1.000000000000000000, 0.000000000000000000 ) ) ;
#117195=FACE_OUTER_BOUND ( 'NONE', #20921, .T. ) ;
#117196=VERTEX_POINT ( 'NONE', #62573 ) ;
#117197=FACE_OUTER_BOUND ( 'NONE', #56092, .T. ) ;
#117198=DIRECTION ( 'NONE',  ( 0.000000000000000000, 0.000000000000000000, -1.000000000000000000 ) ) ;
#117199=EDGE_CURVE ( 'NONE', #98888, #20569, #111662, .T. ) ;
#117200=EDGE_CURVE ( 'NONE', #39357, #105467, #12788, .T. ) ;
#117201=CARTESIAN_POINT ( 'NONE',  ( 6.249999999999932498, 2.500000000000000000, -2.857883832488653741 ) ) ;
#117202=LINE ( 'NONE', #58966, #79955 ) ;
#117203=EDGE_CURVE ( 'NONE', #41353, #51914, #72128, .T. ) ;
#117204=EDGE_CURVE ( 'NONE', #83387, #78182, #52731, .T. ) ;
#117206=AXIS2_PLACEMENT_3D ( 'NONE', #71269, #93500, #22844 ) ;
#117207=ORIENTED_EDGE ( 'NONE', *, *, #31477, .T. ) ;
#117208=CIRCLE ( 'NONE', #48291, 0.06509327318403745899 ) ;
#117209=ORIENTED_EDGE ( 'NONE', *, *, #68476, .F. ) ;
#117210=CARTESIAN_POINT ( 'NONE',  ( -11.44999999999999751, 12.50000000000000000, 2.446380397790835826 ) ) ;
#117211=EDGE_CURVE ( 'NONE', #115271, #30923, #45040, .T. ) ;
#117212=ORIENTED_EDGE ( 'NONE', *, *, #42465, .T. ) ;
#117213=DIRECTION ( 'NONE',  ( 0.000000000000000000, 0.000000000000000000, -1.000000000000000000 ) ) ;
#117214=VERTEX_POINT ( 'NONE', #104413 ) ;
#117215=VERTEX_POINT ( 'NONE', #116795 ) ;
#117216=ORIENTED_EDGE ( 'NONE', *, *, #78991, .F. ) ;
#117217=EDGE_CURVE ( 'NONE', #99388, #29668, #76251, .T. ) ;
#117218=DIRECTION ( 'NONE',  ( -0.000000000000000000, -1.000000000000000000, -0.000000000000000000 ) ) ;
#117220=CARTESIAN_POINT ( 'NONE',  ( 4.349999999999937472, 2.500000000000000000, 6.841600689897072485 ) ) ;
#117221=EDGE_CURVE ( 'NONE', #75789, #11464, #80540, .T. ) ;
#117222=CARTESIAN_POINT ( 'NONE',  ( 6.849999999999927702, 2.500000000000000000, 1.718653347947321386 ) ) ;
#117223=DIRECTION ( 'NONE',  ( 0.000000000000000000, 1.000000000000000000, 0.000000000000000000 ) ) ;
#117224=AXIS2_PLACEMENT_3D ( 'NONE', #91931, #11432, #82110 ) ;
#117225=CARTESIAN_POINT ( 'NONE',  ( 9.999999999999916511, 2.500000000000000000, -0.5928203230275541635 ) ) ;
#117226=DIRECTION ( 'NONE',  ( -0.000000000000000000, -1.000000000000000000, -0.000000000000000000 ) ) ;
#117227=DIRECTION ( 'NONE',  ( -0.000000000000000000, -1.000000000000000000, -0.000000000000000000 ) ) ;
#117228=ORIENTED_EDGE ( 'NONE', *, *, #89731, .T. ) ;
#117229=ADVANCED_FACE ( 'NONE', ( #25195 ), #103518, .T. ) ;
#117230=DIRECTION ( 'NONE',  ( -0.000000000000000000, -1.000000000000000000, -0.000000000000000000 ) ) ;
#117231=ORIENTED_EDGE ( 'NONE', *, *, #14407, .T. ) ;
#117232=ORIENTED_EDGE ( 'NONE', *, *, #38089, .T. ) ;
#117233=ORIENTED_EDGE ( 'NONE', *, *, #30480, .F. ) ;
#117234=ORIENTED_EDGE ( 'NONE', *, *, #91346, .T. ) ;
#117235=LINE ( 'NONE', #57041, #96567 ) ;
#117236=EDGE_LOOP ( 'NONE', ( #96627, #122863, #90708, #2302 ) ) ;
#117237=ORIENTED_EDGE ( 'NONE', *, *, #46908, .T. ) ;
#117238=CARTESIAN_POINT ( 'NONE',  ( -7.900000000000014566, 2.500000000000000000, 0.6928203230275494784 ) ) ;
#117239=DIRECTION ( 'NONE',  ( 0.000000000000000000, 0.000000000000000000, -1.000000000000000000 ) ) ;
#117240=CARTESIAN_POINT ( 'NONE',  ( -0.2000000000000399791, 12.50000000000000000, -4.676537180435977881 ) ) ;
#117241=DIRECTION ( 'NONE',  ( 0.000000000000000000, 0.000000000000000000, 1.000000000000000000 ) ) ;
#117242=AXIS2_PLACEMENT_3D ( 'NONE', #708, #19045, #39385 ) ;
#117243=CARTESIAN_POINT ( 'NONE',  ( -6.650000000000014566, 2.500000000000000000, 5.902370205355745192 ) ) ;
#117244=ORIENTED_EDGE ( 'NONE', *, *, #36538, .F. ) ;
#117245=AXIS2_PLACEMENT_3D ( 'NONE', #21834, #11353, #82688 ) ;
#117246=CONICAL_SURFACE ( 'NONE', #96332, 0.1000000000000000472, 0.003490658503988666988 ) ;
#117248=ORIENTED_EDGE ( 'NONE', *, *, #24188, .T. ) ;
#117249=CARTESIAN_POINT ( 'NONE',  ( 7.049999999999930544, 12.50000000000000000, -6.495190528383302464 ) ) ;
#117250=AXIS2_PLACEMENT_3D ( 'NONE', #122483, #44558, #73364 ) ;
#117251=ORIENTED_EDGE ( 'NONE', *, *, #127160, .F. ) ;
#117252=DIRECTION ( 'NONE',  ( 0.000000000000000000, 0.000000000000000000, 1.000000000000000000 ) ) ;
#117253=VERTEX_POINT ( 'NONE', #5555 ) ;
#117254=ORIENTED_EDGE ( 'NONE', *, *, #28598, .T. ) ;
#117255=LINE ( 'NONE', #109395, #123461 ) ;
#117256=DIRECTION ( 'NONE',  ( 0.000000000000000000, 1.000000000000000000, 0.000000000000000000 ) ) ;
#117258=DIRECTION ( 'NONE',  ( -0.000000000000000000, -1.000000000000000000, -0.000000000000000000 ) ) ;
#117259=DIRECTION ( 'NONE',  ( 0.000000000000000000, 1.000000000000000000, 0.000000000000000000 ) ) ;
#117260=EDGE_CURVE ( 'NONE', #45163, #111163, #124048, .T. ) ;
#117261=CARTESIAN_POINT ( 'NONE',  ( -14.34999999999998543, 2.500000000000000000, -2.411473670974875638 ) ) ;
#117262=EDGE_LOOP ( 'NONE', ( #62598, #12663, #118767, #93866 ) ) ;
#117263=DIRECTION ( 'NONE',  ( -0.000000000000000000, -1.000000000000000000, -0.000000000000000000 ) ) ;
#117264=CARTESIAN_POINT ( 'NONE',  ( 2.899999999999946620, 12.50000000000000000, 0.6928203230275494784 ) ) ;
#117265=LINE ( 'NONE', #116004, #68985 ) ;
#117266=FACE_OUTER_BOUND ( 'NONE', #49559, .T. ) ;
#117267=ADVANCED_FACE ( 'NONE', ( #6193 ), #120247, .T. ) ;
#117268=FACE_OUTER_BOUND ( 'NONE', #38716, .T. ) ;
#117269=ORIENTED_EDGE ( 'NONE', *, *, #9797, .T. ) ;
#117270=AXIS2_PLACEMENT_3D ( 'NONE', #123509, #14825, #33233 ) ;
#117271=ORIENTED_EDGE ( 'NONE', *, *, #40031, .F. ) ;
#117272=CARTESIAN_POINT ( 'NONE',  ( 6.049999999999934097, 12.50000000000000000, -6.148780366869526226 ) ) ;
#117273=ORIENTED_EDGE ( 'NONE', *, *, #5145, .T. ) ;
#117274=LINE ( 'NONE', #67540, #21548 ) ;
#117275=CIRCLE ( 'NONE', #60869, 0.1000000000000002554 ) ;
#117276=CARTESIAN_POINT ( 'NONE',  ( 15.39999999999989200, 2.500000000000000000, -0.6928203230275542523 ) ) ;
#117277=ORIENTED_EDGE ( 'NONE', *, *, #60365, .F. ) ;
#117279=DIRECTION ( 'NONE',  ( 0.000000000000000000, 0.000000000000000000, -1.000000000000000000 ) ) ;
#117280=CARTESIAN_POINT ( 'NONE',  ( -7.499999999999980460, 12.50000000000000000, -4.395220292106239768 ) ) ;
#117281=DIRECTION ( 'NONE',  ( 0.000000000000000000, 0.000000000000000000, 1.000000000000000000 ) ) ;
#117282=ORIENTED_EDGE ( 'NONE', *, *, #2352, .T. ) ;
#117283=CONICAL_SURFACE ( 'NONE', #39965, 0.1000000000000002554, 0.003490658503988666988 ) ;
#117284=DIRECTION ( 'NONE',  ( 0.000000000000000000, 1.000000000000000000, 0.000000000000000000 ) ) ;
#117286=VERTEX_POINT ( 'NONE', #86037 ) ;
#117287=FACE_OUTER_BOUND ( 'NONE', #81903, .T. ) ;
#117288=DIRECTION ( 'NONE',  ( -0.000000000000000000, 1.000000000000000000, -0.000000000000000000 ) ) ;
#117289=FACE_OUTER_BOUND ( 'NONE', #101322, .T. ) ;
#117290=AXIS2_PLACEMENT_3D ( 'NONE', #90096, #58728, #18787 ) ;
#117291=AXIS2_PLACEMENT_3D ( 'NONE', #14760, #54695, #44910 ) ;
#117292=ORIENTED_EDGE ( 'NONE', *, *, #110957, .T. ) ;
#117293=DIRECTION ( 'NONE',  ( -0.000000000000000000, -1.000000000000000000, -0.000000000000000000 ) ) ;
#117294=ORIENTED_EDGE ( 'NONE', *, *, #13674, .F. ) ;
#117295=DIRECTION ( 'NONE',  ( 0.000000000000000000, 1.000000000000000000, 0.000000000000000000 ) ) ;
#117296=DIRECTION ( 'NONE',  ( 0.000000000000000000, 1.000000000000000000, 0.000000000000000000 ) ) ;
#117297=CONICAL_SURFACE ( 'NONE', #14894, 0.1000000000000000472, 0.003490658503988666988 ) ;
#117298=CARTESIAN_POINT ( 'NONE',  ( -1.250000000000001110, 12.50000000000000000, -6.495190528383302464 ) ) ;
#117299=EDGE_LOOP ( 'NONE', ( #11024, #90247 ) ) ;
#117300=DIRECTION ( 'NONE',  ( 0.000000000000000000, -0.9999939076577903929, 0.003490651415223739937 ) ) ;
#117301=CARTESIAN_POINT ( 'NONE',  ( -10.80000000000000071, 2.500000000000000000, 0.09999999999999772959 ) ) ;
#117302=CIRCLE ( 'NONE', #33806, 0.1000000000000000472 ) ;
#117303=CIRCLE ( 'NONE', #19035, 0.06509327318403745899 ) ;
#117305=ORIENTED_EDGE ( 'NONE', *, *, #19733, .F. ) ;
#117306=LINE ( 'NONE', #47324, #2969 ) ;
#117307=ADVANCED_FACE ( 'NONE', ( #15364 ), #70068, .T. ) ;
#117308=VERTEX_POINT ( 'NONE', #46135 ) ;
#117309=DIRECTION ( 'NONE',  ( 0.000000000000000000, 1.000000000000000000, 0.000000000000000000 ) ) ;
#117310=ORIENTED_EDGE ( 'NONE', *, *, #115651, .F. ) ;
#117311=CARTESIAN_POINT ( 'NONE',  ( -6.050000000000022027, 12.50000000000000000, -6.148780366869526226 ) ) ;
#117312=DIRECTION ( 'NONE',  ( 0.000000000000000000, 1.000000000000000000, 0.000000000000000000 ) ) ;
#117313=VERTEX_POINT ( 'NONE', #106970 ) ;
#117314=EDGE_CURVE ( 'NONE', #46749, #92080, #32444, .T. ) ;
#117315=ORIENTED_EDGE ( 'NONE', *, *, #127267, .F. ) ;
#117316=DIRECTION ( 'NONE',  ( 0.000000000000000000, 0.000000000000000000, 1.000000000000000000 ) ) ;
#117317=LINE ( 'NONE', #27669, #109085 ) ;
#117318=ORIENTED_EDGE ( 'NONE', *, *, #80617, .T. ) ;
#117319=DIRECTION ( 'NONE',  ( -0.000000000000000000, 1.000000000000000000, -0.000000000000000000 ) ) ;
#117320=CARTESIAN_POINT ( 'NONE',  ( 1.849999999999950573, 2.500000000000000000, 2.511473670974873507 ) ) ;
#117321=AXIS2_PLACEMENT_3D ( 'NONE', #5851, #96817, #76548 ) ;
#117322=CARTESIAN_POINT ( 'NONE',  ( 15.79999999999989058, 12.50000000000000000, -2.385244779468109755E-15 ) ) ;
#117325=VECTOR ( 'NONE', #29695, 1000.000000000000000 ) ;
#117326=CARTESIAN_POINT ( 'NONE',  ( -4.150000000000027889, 2.500000000000000000, -7.088010851410853519 ) ) ;
#117327=FACE_OUTER_BOUND ( 'NONE', #16363, .T. ) ;
#117328=AXIS2_PLACEMENT_3D ( 'NONE', #13642, #2524, #43782 ) ;
#117329=ORIENTED_EDGE ( 'NONE', *, *, #44430, .T. ) ;
#117330=EDGE_CURVE ( 'NONE', #35601, #34064, #1099, .T. ) ;
#117331=ORIENTED_EDGE ( 'NONE', *, *, #70404, .F. ) ;
#117332=VERTEX_POINT ( 'NONE', #106345 ) ;
#117333=ORIENTED_EDGE ( 'NONE', *, *, #47482, .F. ) ;
#117334=FACE_OUTER_BOUND ( 'NONE', #1951, .T. ) ;
#117335=DIRECTION ( 'NONE',  ( -0.000000000000000000, -1.000000000000000000, -0.000000000000000000 ) ) ;
#117336=CONICAL_SURFACE ( 'NONE', #94383, 0.1000000000000000472, 0.003490658503988666988 ) ;
#117337=DIRECTION ( 'NONE',  ( -0.000000000000000000, 1.000000000000000000, -0.000000000000000000 ) ) ;
#117338=ORIENTED_EDGE ( 'NONE', *, *, #64193, .T. ) ;
#117339=FACE_BOUND ( 'NONE', #43183, .T. ) ;
#117340=ORIENTED_EDGE ( 'NONE', *, *, #122780, .F. ) ;
#117341=CARTESIAN_POINT ( 'NONE',  ( -6.250000000000017764, 12.50000000000000000, 7.188010851410848723 ) ) ;
#117342=CARTESIAN_POINT ( 'NONE',  ( -5.850000000000018296, 2.500000000000000000, 2.957883832488649389 ) ) ;
#117343=CARTESIAN_POINT ( 'NONE',  ( -6.900000000000019007, 12.50000000000000000, -0.3464101615137783474 ) ) ;
#117344=ADVANCED_FACE ( 'NONE', ( #34409 ), #90992, .T. ) ;
#117345=DIRECTION ( 'NONE',  ( 0.000000000000000000, -0.9999939076577903929, 0.003490651415223739937 ) ) ;
#117346=CARTESIAN_POINT ( 'NONE',  ( 17.49862860983209600, -2.500000000000000000, 4.081131818001135336 ) ) ;
#117347=CARTESIAN_POINT ( 'NONE',  ( 14.59999999999989484, 2.500000000000000000, 0.7928203230275495672 ) ) ;
#117348=DIRECTION ( 'NONE',  ( 0.000000000000000000, 0.000000000000000000, 1.000000000000000000 ) ) ;
#117349=DIRECTION ( 'NONE',  ( -0.000000000000000000, -1.000000000000000000, -0.000000000000000000 ) ) ;
#117350=EDGE_CURVE ( 'NONE', #44383, #41372, #84118, .T. ) ;
#117351=ADVANCED_FACE ( 'NONE', ( #74317 ), #28303, .T. ) ;
#117352=CARTESIAN_POINT ( 'NONE',  ( -0.6000000000000388356, 2.500000000000000000, 3.983716857408420964 ) ) ;
#117353=ADVANCED_FACE ( 'NONE', ( #56580 ), #105576, .T. ) ;
#117354=EDGE_CURVE ( 'NONE', #14513, #54407, #11560, .T. ) ;
#117355=CARTESIAN_POINT ( 'NONE',  ( 6.899999999999926636, 2.500000000000000000, -0.4464101615137782142 ) ) ;
#117356=ORIENTED_EDGE ( 'NONE', *, *, #14086, .T. ) ;
#117357=EDGE_LOOP ( 'NONE', ( #18134, #88108, #95188, #85020 ) ) ;
#117358=EDGE_LOOP ( 'NONE', ( #73799, #7291 ) ) ;
#117360=DIRECTION ( 'NONE',  ( 0.000000000000000000, 1.000000000000000000, 0.000000000000000000 ) ) ;
#117361=EDGE_CURVE ( 'NONE', #23570, #32403, #4906, .T. ) ;
#117362=DIRECTION ( 'NONE',  ( 0.000000000000000000, 0.000000000000000000, -1.000000000000000000 ) ) ;
#117363=EDGE_CURVE ( 'NONE', #113534, #76503, #127919, .T. ) ;
#117364=ORIENTED_EDGE ( 'NONE', *, *, #63441, .F. ) ;
#117365=VERTEX_POINT ( 'NONE', #129241 ) ;
#117366=ORIENTED_EDGE ( 'NONE', *, *, #15042, .F. ) ;
#117367=DIRECTION ( 'NONE',  ( -4.274815082592931898E-19, -0.9999939076577903929, -0.003490651415223739937 ) ) ;
#117368=AXIS2_PLACEMENT_3D ( 'NONE', #3803, #24736, #43754 ) ;
#117369=CONICAL_SURFACE ( 'NONE', #12820, 0.1000000000000002554, 0.003490658503988666988 ) ;
#117370=EDGE_CURVE ( 'NONE', #8727, #43078, #84731, .T. ) ;
#117371=EDGE_CURVE ( 'NONE', #114782, #45293, #101463, .T. ) ;
#117372=CARTESIAN_POINT ( 'NONE',  ( -3.749999999999991118, 2.500000000000000000, -2.165063509461101710 ) ) ;
#117373=CARTESIAN_POINT ( 'NONE',  ( 3.549999999999943867, 12.50000000000000000, -1.883746621131363597 ) ) ;
#117374=CARTESIAN_POINT ( 'NONE',  ( 0.6499999999999561684, 2.500000000000000000, -1.818653347947325916 ) ) ;
#117375=CARTESIAN_POINT ( 'NONE',  ( 8.099999999999921485, 12.50000000000000000, 0.3464101615137735735 ) ) ;
#117376=DIRECTION ( 'NONE',  ( 0.000000000000000000, 1.000000000000000000, 0.000000000000000000 ) ) ;
#117377=ADVANCED_FACE ( 'NONE', ( #58551 ), #49159, .T. ) ;
#117378=VERTEX_POINT ( 'NONE', #117420 ) ;
#117379=AXIS2_PLACEMENT_3D ( 'NONE', #11717, #121668, #22209 ) ;
#117380=EDGE_CURVE ( 'NONE', #104514, #16978, #68350, .T. ) ;
#117381=VECTOR ( 'NONE', #125633, 1000.000000000000000 ) ;
#117382=DIRECTION ( 'NONE',  ( -0.000000000000000000, 1.000000000000000000, -0.000000000000000000 ) ) ;
#117383=ORIENTED_EDGE ( 'NONE', *, *, #57166, .T. ) ;
#117384=EDGE_LOOP ( 'NONE', ( #93762, #36410 ) ) ;
#117386=EDGE_LOOP ( 'NONE', ( #19575, #88059, #51197, #88148 ) ) ;
#117387=CARTESIAN_POINT ( 'NONE',  ( 9.799999999999915445, 2.500000000000000000, -4.676537180435977881 ) ) ;
#117388=ORIENTED_EDGE ( 'NONE', *, *, #59188, .T. ) ;
#117389=ORIENTED_EDGE ( 'NONE', *, *, #108190, .F. ) ;
#117390=CIRCLE ( 'NONE', #54708, 0.06509327318403745899 ) ;
#117391=DIRECTION ( 'NONE',  ( -0.000000000000000000, 1.000000000000000000, -0.000000000000000000 ) ) ;
#117392=VECTOR ( 'NONE', #126534, 1000.000000000000000 ) ;
#117393=DIRECTION ( 'NONE',  ( -4.274815082592931898E-19, -0.9999939076577903929, -0.003490651415223739937 ) ) ;
#117394=DIRECTION ( 'NONE',  ( 0.000000000000000000, -0.9999939076577903929, 0.003490651415223739937 ) ) ;
#117395=CARTESIAN_POINT ( 'NONE',  ( -8.150000000000012790, 2.500000000000000000, -1.918653347947326004 ) ) ;
#117396=CONICAL_SURFACE ( 'NONE', #60984, 0.1000000000000002554, 0.003490658503988666988 ) ;
#117397=DIRECTION ( 'NONE',  ( 0.000000000000000000, -0.9999939076577903929, 0.003490651415223739937 ) ) ;
#117398=CIRCLE ( 'NONE', #25476, 0.06509327318403745899 ) ;
#117399=EDGE_LOOP ( 'NONE', ( #95203, #43940 ) ) ;
#117400=DIRECTION ( 'NONE',  ( 0.000000000000000000, -0.9999939076577903929, 0.003490651415223739937 ) ) ;
#117401=ORIENTED_EDGE ( 'NONE', *, *, #94030, .T. ) ;
#117403=VERTEX_POINT ( 'NONE', #98441 ) ;
#117405=CIRCLE ( 'NONE', #17138, 0.06509327318403745899 ) ;
#117406=CONICAL_SURFACE ( 'NONE', #33807, 0.1000000000000000056, 0.003490658503988666988 ) ;
#117407=DIRECTION ( 'NONE',  ( -0.000000000000000000, 1.000000000000000000, -0.000000000000000000 ) ) ;
#117408=ORIENTED_EDGE ( 'NONE', *, *, #4933, .T. ) ;
#117409=FACE_OUTER_BOUND ( 'NONE', #93902, .T. ) ;
#117410=DIRECTION ( 'NONE',  ( -0.000000000000000000, -1.000000000000000000, -0.000000000000000000 ) ) ;
#117411=ORIENTED_EDGE ( 'NONE', *, *, #43148, .F. ) ;
#117412=EDGE_CURVE ( 'NONE', #66216, #96385, #38793, .T. ) ;
#117413=CARTESIAN_POINT ( 'NONE',  ( 8.949999999999919353, 2.500000000000000000, -6.148780366869526226 ) ) ;
#117414=EDGE_CURVE ( 'NONE', #109336, #125197, #17825, .T. ) ;
#117415=ORIENTED_EDGE ( 'NONE', *, *, #52507, .F. ) ;
#117416=ORIENTED_EDGE ( 'NONE', *, *, #72169, .F. ) ;
#117417=DIRECTION ( 'NONE',  ( 0.000000000000000000, 0.000000000000000000, -1.000000000000000000 ) ) ;
#117418=DIRECTION ( 'NONE',  ( 0.000000000000000000, 0.000000000000000000, 1.000000000000000000 ) ) ;
#117420=CARTESIAN_POINT ( 'NONE',  ( -15.59999999999998010, 2.500000000000000000, 0.4464101615137759382 ) ) ;
#117422=DIRECTION ( 'NONE',  ( -4.274815082592931898E-19, -0.9999939076577903929, -0.003490651415223739937 ) ) ;
#117423=AXIS2_PLACEMENT_3D ( 'NONE', #115667, #26021, #67186 ) ;
#117424=AXIS2_PLACEMENT_3D ( 'NONE', #85236, #15841, #34222 ) ;
#117425=ORIENTED_EDGE ( 'NONE', *, *, #44258, .T. ) ;
#117426=CARTESIAN_POINT ( 'NONE',  ( -5.800000000000018474, 12.50000000000000000, 4.330127018922196314 ) ) ;
#117427=CARTESIAN_POINT ( 'NONE',  ( -11.44999999999999929, 2.500000000000000000, -1.718653347947322052 ) ) ;
#117428=AXIS2_PLACEMENT_3D ( 'NONE', #115962, #127084, #46563 ) ;
#117430=AXIS2_PLACEMENT_3D ( 'NONE', #7583, #58644, #37071 ) ;
#117431=CONICAL_SURFACE ( 'NONE', #52717, 0.1000000000000000472, 0.003490658503988666988 ) ;
#117432=CARTESIAN_POINT ( 'NONE',  ( -5.000000000000022204, 12.50000000000000000, -0.6928203230275541413 ) ) ;
#117433=CARTESIAN_POINT ( 'NONE',  ( -0.8500000000000382805, 12.50000000000000000, -1.472243186433550122 ) ) ;
#117434=CARTESIAN_POINT ( 'NONE',  ( -1.250000000000035749, 2.500000000000000000, -2.857883832488653741 ) ) ;
#117436=CARTESIAN_POINT ( 'NONE',  ( 8.949999999999917577, 2.500000000000000000, -2.511473670974877948 ) ) ;
#117437=ORIENTED_EDGE ( 'NONE', *, *, #7895, .T. ) ;
#117438=AXIS2_PLACEMENT_3D ( 'NONE', #41720, #81618, #111730 ) ;
#117439=CARTESIAN_POINT ( 'NONE',  ( -12.89999999999999325, 2.500000000000000000, -3.637306695894647390 ) ) ;
#117441=EDGE_LOOP ( 'NONE', ( #71250, #101791 ) ) ;
#117442=DIRECTION ( 'NONE',  ( -0.000000000000000000, 1.000000000000000000, -0.000000000000000000 ) ) ;
#117443=ADVANCED_FACE ( 'NONE', ( #87968 ), #108276, .T. ) ;
#117444=ORIENTED_EDGE ( 'NONE', *, *, #38950, .T. ) ;
#117445=VERTEX_POINT ( 'NONE', #48728 ) ;
#117446=DIRECTION ( 'NONE',  ( 0.000000000000000000, 1.000000000000000000, 0.000000000000000000 ) ) ;
#117447=VERTEX_POINT ( 'NONE', #27773 ) ;
#117448=CARTESIAN_POINT ( 'NONE',  ( -1.650000000000034328, 2.500000000000000000, -7.288010851410854585 ) ) ;
#117449=DIRECTION ( 'NONE',  ( 0.000000000000000000, 0.000000000000000000, 1.000000000000000000 ) ) ;
#117450=CARTESIAN_POINT ( 'NONE',  ( 4.999999999999936939, 12.50000000000000000, -0.7579135962115916003 ) ) ;
#117451=CONICAL_SURFACE ( 'NONE', #100748, 0.09999999999999982514, 0.003490658503988666988 ) ;
#117452=ORIENTED_EDGE ( 'NONE', *, *, #129559, .T. ) ;
#117453=AXIS2_PLACEMENT_3D ( 'NONE', #47266, #114692, #87164 ) ;
#117454=DIRECTION ( 'NONE',  ( -0.000000000000000000, 1.000000000000000000, -0.000000000000000000 ) ) ;
#117455=CARTESIAN_POINT ( 'NONE',  ( 9.799999999999917222, 2.500000000000000000, 0.3464101615137735735 ) ) ;
#117456=ORIENTED_EDGE ( 'NONE', *, *, #32552, .T. ) ;
#117457=EDGE_CURVE ( 'NONE', #67849, #35226, #47096, .T. ) ;
#117458=DIRECTION ( 'NONE',  ( 0.000000000000000000, 1.000000000000000000, 0.000000000000000000 ) ) ;
#117459=LINE ( 'NONE', #21721, #59305 ) ;
#117460=EDGE_CURVE ( 'NONE', #119760, #127429, #57907, .T. ) ;
#117461=AXIS2_PLACEMENT_3D ( 'NONE', #13643, #93508, #3833 ) ;
#117462=ORIENTED_EDGE ( 'NONE', *, *, #119476, .T. ) ;
#117463=CIRCLE ( 'NONE', #56836, 0.06509327318403745899 ) ;
#117464=AXIS2_PLACEMENT_3D ( 'NONE', #112316, #4915, #122775 ) ;
#117466=ORIENTED_EDGE ( 'NONE', *, *, #33016, .F. ) ;
#117467=DIRECTION ( 'NONE',  ( 0.000000000000000000, 0.000000000000000000, -1.000000000000000000 ) ) ;
#117468=LINE ( 'NONE', #127968, #81276 ) ;
#117469=CARTESIAN_POINT ( 'NONE',  ( 14.14999999999989377, 2.500000000000000000, -2.857883832488653741 ) ) ;
#117471=ADVANCED_FACE ( 'NONE', ( #37620 ), #59196, .T. ) ;
#117472=FACE_BOUND ( 'NONE', #45107, .T. ) ;
#117473=ORIENTED_EDGE ( 'NONE', *, *, #36262, .F. ) ;
#117474=DIRECTION ( 'NONE',  ( 0.000000000000000000, -0.000000000000000000, 1.000000000000000000 ) ) ;
#117475=DIRECTION ( 'NONE',  ( 0.000000000000000000, 0.000000000000000000, 1.000000000000000000 ) ) ;
#117476=AXIS2_PLACEMENT_3D ( 'NONE', #3985, #24284, #64198 ) ;
#117477=VERTEX_POINT ( 'NONE', #67699 ) ;
#117478=AXIS2_PLACEMENT_3D ( 'NONE', #7381, #47332, #42014 ) ;
#117480=CIRCLE ( 'NONE', #127980, 0.06509327318403745899 ) ;
#117481=AXIS2_PLACEMENT_3D ( 'NONE', #77340, #26957, #89100 ) ;
#117482=CIRCLE ( 'NONE', #19302, 0.1000000000000002554 ) ;
#117483=FACE_OUTER_BOUND ( 'NONE', #38713, .T. ) ;
#117484=DIRECTION ( 'NONE',  ( 0.000000000000000000, 0.000000000000000000, -1.000000000000000000 ) ) ;
#117485=DIRECTION ( 'NONE',  ( 0.000000000000000000, 0.000000000000000000, 1.000000000000000000 ) ) ;
#117486=AXIS2_PLACEMENT_3D ( 'NONE', #9819, #80509, #81148 ) ;
#117487=DIRECTION ( 'NONE',  ( -0.000000000000000000, -1.000000000000000000, -0.000000000000000000 ) ) ;
#117488=ORIENTED_EDGE ( 'NONE', *, *, #79845, .T. ) ;
#117489=AXIS2_PLACEMENT_3D ( 'NONE', #87734, #38005, #89685 ) ;
#117490=ORIENTED_EDGE ( 'NONE', *, *, #93575, .F. ) ;
#117491=EDGE_LOOP ( 'NONE', ( #84032, #128171, #125258, #25273 ) ) ;
#117492=EDGE_LOOP ( 'NONE', ( #76053, #70321, #33732, #38083 ) ) ;
#117493=EDGE_LOOP ( 'NONE', ( #6526, #116272, #188, #118350 ) ) ;
#117494=DIRECTION ( 'NONE',  ( -0.000000000000000000, -1.000000000000000000, -0.000000000000000000 ) ) ;
#117495=DIRECTION ( 'NONE',  ( 0.000000000000000000, 0.000000000000000000, -1.000000000000000000 ) ) ;
#117496=ORIENTED_EDGE ( 'NONE', *, *, #86774, .F. ) ;
#117497=FACE_BOUND ( 'NONE', #69874, .T. ) ;
#117498=CARTESIAN_POINT ( 'NONE',  ( -11.04999999999999893, 12.50000000000000000, 1.883746621131358934 ) ) ;
#117499=EDGE_CURVE ( 'NONE', #41725, #128844, #55398, .T. ) ;
#117500=CARTESIAN_POINT ( 'NONE',  ( -3.750000000000026201, 2.500000000000000000, 5.802370205355744659 ) ) ;
#117501=DIRECTION ( 'NONE',  ( 0.000000000000000000, -0.9999939076577903929, 0.003490651415223739937 ) ) ;
#117502=CARTESIAN_POINT ( 'NONE',  ( -1.250000000000036193, 2.500000000000000000, 5.802370205355744659 ) ) ;
#117503=ADVANCED_FACE ( 'NONE', ( #107640 ), #19903, .T. ) ;
#117504=DIRECTION ( 'NONE',  ( 0.000000000000000000, 0.000000000000000000, -1.000000000000000000 ) ) ;
#117505=ORIENTED_EDGE ( 'NONE', *, *, #126901, .F. ) ;
#117506=LINE ( 'NONE', #1465, #17980 ) ;
#117507=EDGE_CURVE ( 'NONE', #71451, #86508, #36637, .T. ) ;
#117508=ORIENTED_EDGE ( 'NONE', *, *, #121368, .T. ) ;
#117509=ORIENTED_EDGE ( 'NONE', *, *, #324, .T. ) ;
#117510=CONICAL_SURFACE ( 'NONE', #77828, 0.1000000000000002554, 0.003490658503988666988 ) ;
#117511=ORIENTED_EDGE ( 'NONE', *, *, #36901, .T. ) ;
#117512=EDGE_CURVE ( 'NONE', #22290, #90888, #42997, .T. ) ;
#117513=DIRECTION ( 'NONE',  ( 0.000000000000000000, 0.000000000000000000, -1.000000000000000000 ) ) ;
#117514=VECTOR ( 'NONE', #67, 1000.000000000000000 ) ;
#117515=DIRECTION ( 'NONE',  ( 0.000000000000000000, 0.000000000000000000, 1.000000000000000000 ) ) ;
#117516=EDGE_CURVE ( 'NONE', #72858, #30037, #19992, .T. ) ;
#117518=EDGE_CURVE ( 'NONE', #63031, #2959, #10081, .T. ) ;
#117519=ORIENTED_EDGE ( 'NONE', *, *, #101946, .F. ) ;
#117520=CARTESIAN_POINT ( 'NONE',  ( 10.87377556668899814, 2.500000000000640821, -8.986829607521531926 ) ) ;
#117521=EDGE_CURVE ( 'NONE', #34246, #28046, #5398, .T. ) ;
#117522=DIRECTION ( 'NONE',  ( 0.000000000000000000, 0.000000000000000000, -1.000000000000000000 ) ) ;
#117523=AXIS2_PLACEMENT_3D ( 'NONE', #32785, #11819, #62864 ) ;
#117524=AXIS2_PLACEMENT_3D ( 'NONE', #52273, #103945, #3171 ) ;
#117525=AXIS2_PLACEMENT_3D ( 'NONE', #102752, #34025, #54309 ) ;
#117526=PLANE ( 'NONE',  #28618 ) ;
#117527=EDGE_CURVE ( 'NONE', #61622, #76508, #60491, .T. ) ;
#117529=CARTESIAN_POINT ( 'NONE',  ( 2.699999999999946443, 2.500000000000000000, -3.983716857408426293 ) ) ;
#117530=DIRECTION ( 'NONE',  ( 0.000000000000000000, 1.000000000000000000, 0.000000000000000000 ) ) ;
#117531=AXIS2_PLACEMENT_3D ( 'NONE', #118036, #108853, #68287 ) ;
#117532=AXIS2_PLACEMENT_3D ( 'NONE', #16920, #85050, #45791 ) ;
#117533=CARTESIAN_POINT ( 'NONE',  ( 8.549999999999920774, 2.500000000000000000, 6.248780366869521430 ) ) ;
#117534=EDGE_LOOP ( 'NONE', ( #124393, #125456 ) ) ;
#117535=DIRECTION ( 'NONE',  ( -4.274815082592931898E-19, -0.9999939076577903929, -0.003490651415223739937 ) ) ;
#117536=ADVANCED_FACE ( 'NONE', ( #102333 ), #31037, .T. ) ;
#117537=CIRCLE ( 'NONE', #88297, 0.09999999999999982514 ) ;
#117538=VERTEX_POINT ( 'NONE', #51316 ) ;
#117539=ORIENTED_EDGE ( 'NONE', *, *, #105157, .F. ) ;
#117540=CARTESIAN_POINT ( 'NONE',  ( -1.450000000000035483, 12.50000000000000000, 1.818653347947321475 ) ) ;
#117541=DIRECTION ( 'NONE',  ( -0.000000000000000000, -1.000000000000000000, -0.000000000000000000 ) ) ;
#117542=DIRECTION ( 'NONE',  ( -0.000000000000000000, -1.000000000000000000, -0.000000000000000000 ) ) ;
#117543=EDGE_LOOP ( 'NONE', ( #42094, #124747, #21839, #21734 ) ) ;
#117544=VERTEX_POINT ( 'NONE', #123258 ) ;
#117545=VECTOR ( 'NONE', #127319, 1000.000000000000000 ) ;
#117546=CARTESIAN_POINT ( 'NONE',  ( -1.850000000000033396, 12.50000000000000000, -2.511473670974877948 ) ) ;
#117547=CARTESIAN_POINT ( 'NONE',  ( 4.599999999999937472, 2.500000000000000000, 0.6928203230275494784 ) ) ;
#117548=CARTESIAN_POINT ( 'NONE',  ( -10.84999999999999964, 2.500000000000000000, 5.802370205355744659 ) ) ;
#117549=ORIENTED_EDGE ( 'NONE', *, *, #64170, .T. ) ;
#117550=ORIENTED_EDGE ( 'NONE', *, *, #127785, .T. ) ;
#117551=DIRECTION ( 'NONE',  ( -0.000000000000000000, -1.000000000000000000, -0.000000000000000000 ) ) ;
#117552=ORIENTED_EDGE ( 'NONE', *, *, #71448, .F. ) ;
#117553=DIRECTION ( 'NONE',  ( 0.000000000000000000, 0.000000000000000000, 1.000000000000000000 ) ) ;
#117554=AXIS2_PLACEMENT_3D ( 'NONE', #22415, #72788, #121879 ) ;
#117556=ORIENTED_EDGE ( 'NONE', *, *, #50221, .T. ) ;
#117557=DIRECTION ( 'NONE',  ( 0.000000000000000000, 0.000000000000000000, 1.000000000000000000 ) ) ;
#117558=DIRECTION ( 'NONE',  ( 0.000000000000000000, -0.000000000000000000, 1.000000000000000000 ) ) ;
#117559=FACE_OUTER_BOUND ( 'NONE', #81379, .T. ) ;
#117560=CARTESIAN_POINT ( 'NONE',  ( -4.200000000000025935, 2.500000000000000000, 4.230127018922196669 ) ) ;
#117561=VECTOR ( 'NONE', #104452, 1000.000000000000000 ) ;
#117562=ORIENTED_EDGE ( 'NONE', *, *, #129403, .F. ) ;
#117563=AXIS2_PLACEMENT_3D ( 'NONE', #78810, #117391, #8736 ) ;
#117564=AXIS2_PLACEMENT_3D ( 'NONE', #44629, #22433, #124481 ) ;
#117565=DIRECTION ( 'NONE',  ( -0.000000000000000000, -1.000000000000000000, -0.000000000000000000 ) ) ;
#117566=CIRCLE ( 'NONE', #75729, 0.1000000000000000472 ) ;
#117567=EDGE_CURVE ( 'NONE', #59434, #90074, #32327, .T. ) ;
#117568=EDGE_LOOP ( 'NONE', ( #17010, #35975 ) ) ;
#117569=ORIENTED_EDGE ( 'NONE', *, *, #38060, .T. ) ;
#117570=LINE ( 'NONE', #88788, #41610 ) ;
#117572=PLANE ( 'NONE',  #7113 ) ;
#117573=DIRECTION ( 'NONE',  ( 0.000000000000000000, 0.000000000000000000, 1.000000000000000000 ) ) ;
#117574=AXIS2_PLACEMENT_3D ( 'NONE', #79202, #119749, #81131 ) ;
#117575=FACE_OUTER_BOUND ( 'NONE', #27723, .T. ) ;
#117576=DIRECTION ( 'NONE',  ( -0.000000000000000000, 1.000000000000000000, -0.000000000000000000 ) ) ;
#117577=VECTOR ( 'NONE', #59601, 1000.000000000000000 ) ;
#117578=EDGE_CURVE ( 'NONE', #58093, #84838, #1200, .T. ) ;
#117579=CARTESIAN_POINT ( 'NONE',  ( 13.74999999999989875, 2.500000000000000000, 1.572243186433545548 ) ) ;
#117580=CONICAL_SURFACE ( 'NONE', #75742, 0.1000000000000000056, 0.003490658503988666988 ) ;
#117581=CARTESIAN_POINT ( 'NONE',  ( -12.89999999999999147, 2.500000000000000000, -4.922947341949750921 ) ) ;
#117582=AXIS2_PLACEMENT_3D ( 'NONE', #43880, #92970, #3293 ) ;
#117583=AXIS2_PLACEMENT_3D ( 'NONE', #11785, #2596, #121099 ) ;
#117584=DIRECTION ( 'NONE',  ( 0.000000000000000000, 0.000000000000000000, 1.000000000000000000 ) ) ;
#117585=CIRCLE ( 'NONE', #113413, 0.1000000000000000472 ) ;
#117586=DIRECTION ( 'NONE',  ( 0.000000000000000000, 0.000000000000000000, -1.000000000000000000 ) ) ;
#117587=AXIS2_PLACEMENT_3D ( 'NONE', #81004, #12878, #60093 ) ;
#117588=ORIENTED_EDGE ( 'NONE', *, *, #30238, .T. ) ;
#117589=DIRECTION ( 'NONE',  ( -0.000000000000000000, 1.000000000000000000, -0.000000000000000000 ) ) ;
#117590=LINE ( 'NONE', #58705, #81399 ) ;
#117592=CARTESIAN_POINT ( 'NONE',  ( -10.80000000000000071, 2.500000000000000000, -2.276824562219559311E-15 ) ) ;
#117593=DIRECTION ( 'NONE',  ( 0.000000000000000000, 0.000000000000000000, 1.000000000000000000 ) ) ;
#117594=EDGE_LOOP ( 'NONE', ( #13391, #109390 ) ) ;
#117595=CARTESIAN_POINT ( 'NONE',  ( 13.74999999999989875, 2.500000000000000000, 1.472243186433545459 ) ) ;
#117596=FACE_OUTER_BOUND ( 'NONE', #4359, .T. ) ;
#117597=DIRECTION ( 'NONE',  ( 0.000000000000000000, 1.000000000000000000, 0.000000000000000000 ) ) ;
#117598=ORIENTED_EDGE ( 'NONE', *, *, #71889, .T. ) ;
#117599=AXIS2_PLACEMENT_3D ( 'NONE', #79941, #119867, #32801 ) ;
#117600=ORIENTED_EDGE ( 'NONE', *, *, #127421, .T. ) ;
#117601=EDGE_CURVE ( 'NONE', #65687, #81044, #50646, .T. ) ;
#117602=ORIENTED_EDGE ( 'NONE', *, *, #121051, .T. ) ;
#117603=ORIENTED_EDGE ( 'NONE', *, *, #13656, .T. ) ;
#117604=ORIENTED_EDGE ( 'NONE', *, *, #71344, .F. ) ;
#117605=CARTESIAN_POINT ( 'NONE',  ( -6.450000000000019718, 12.50000000000000000, -1.818653347947326138 ) ) ;
#117606=CIRCLE ( 'NONE', #75772, 0.06509327318403745899 ) ;
#117607=DIRECTION ( 'NONE',  ( 0.000000000000000000, 1.000000000000000000, 0.000000000000000000 ) ) ;
#117608=DIRECTION ( 'NONE',  ( 0.000000000000000000, 1.000000000000000000, 0.000000000000000000 ) ) ;
#117609=DIRECTION ( 'NONE',  ( -0.000000000000000000, -1.000000000000000000, -0.000000000000000000 ) ) ;
#117610=EDGE_CURVE ( 'NONE', #125433, #125134, #24191, .T. ) ;
#117611=CONICAL_SURFACE ( 'NONE', #121751, 0.1000000000000002554, 0.003490658503988666988 ) ;
#117612=ORIENTED_EDGE ( 'NONE', *, *, #38790, .T. ) ;
#117613=CIRCLE ( 'NONE', #59072, 0.1000000000000000472 ) ;
#117614=CIRCLE ( 'NONE', #119695, 0.09999999999999982514 ) ;
#117615=DIRECTION ( 'NONE',  ( -0.000000000000000000, 1.000000000000000000, -0.000000000000000000 ) ) ;
#117616=VECTOR ( 'NONE', #101638, 1000.000000000000000 ) ;
#117617=VERTEX_POINT ( 'NONE', #21183 ) ;
#117618=CARTESIAN_POINT ( 'NONE',  ( 21.24754738303276369, -0.7337760880902376437, -4.182111650399355618 ) ) ;
#117619=CARTESIAN_POINT ( 'NONE',  ( -4.150000000000024336, 12.50000000000000000, -2.857883832488653741 ) ) ;
#117620=VECTOR ( 'NONE', #88701, 1000.000000000000000 ) ;
#117621=ADVANCED_FACE ( 'NONE', ( #1537 ), #38896, .T. ) ;
#117622=CARTESIAN_POINT ( 'NONE',  ( 21.24754738303277435, 0.7337760880902391980, 4.182111650399362723 ) ) ;
#117623=CONICAL_SURFACE ( 'NONE', #90442, 0.1000000000000000472, 0.003490658503988666988 ) ;
#117624=FACE_OUTER_BOUND ( 'NONE', #46129, .T. ) ;
#117625=CARTESIAN_POINT ( 'NONE',  ( -1.250000000000036193, 2.500000000000000000, 1.372243186433545370 ) ) ;
#117626=ADVANCED_FACE ( 'NONE', ( #41502 ), #101037, .T. ) ;
#117627=CIRCLE ( 'NONE', #42361, 0.1000000000000000472 ) ;
#117628=VERTEX_POINT ( 'NONE', #61775 ) ;
#117629=EDGE_LOOP ( 'NONE', ( #94150, #26574, #55146, #67156 ) ) ;
#117630=ADVANCED_FACE ( 'NONE', ( #12007 ), #97343, .T. ) ;
#117631=ORIENTED_EDGE ( 'NONE', *, *, #110256, .T. ) ;
#117632=ORIENTED_EDGE ( 'NONE', *, *, #73089, .T. ) ;
#117633=PLANE ( 'NONE',  #25197 ) ;
#117634=CARTESIAN_POINT ( 'NONE',  ( 32.27737261616376685, 1.406459146825700390, 4.686451385765966648 ) ) ;
#117635=DIRECTION ( 'NONE',  ( 0.000000000000000000, 0.000000000000000000, 1.000000000000000000 ) ) ;
#117636=EDGE_CURVE ( 'NONE', #96595, #42755, #72869, .T. ) ;
#117637=FACE_BOUND ( 'NONE', #91265, .T. ) ;
#117638=DIRECTION ( 'NONE',  ( 0.000000000000000000, 1.000000000000000000, 0.000000000000000000 ) ) ;
#117640=CARTESIAN_POINT ( 'NONE',  ( -2.500000000000031086, 2.500000000000000000, 3.637306695894644726 ) ) ;
#117641=CARTESIAN_POINT ( 'NONE',  ( 6.849999999999930367, 2.500000000000000000, -6.148780366869526226 ) ) ;
#117643=CARTESIAN_POINT ( 'NONE',  ( -3.350000000000028955, 12.50000000000000000, 7.253104124594885960 ) ) ;
#117644=FACE_OUTER_BOUND ( 'NONE', #101968, .T. ) ;
#117645=CIRCLE ( 'NONE', #61250, 0.06509327318403745899 ) ;
#117646=VECTOR ( 'NONE', #11429, 1000.000000000000000 ) ;
#117647=AXIS2_PLACEMENT_3D ( 'NONE', #83876, #124465, #15119 ) ;
#117648=CARTESIAN_POINT ( 'NONE',  ( -7.700000000000014388, 2.500000000000000000, -0.3464101615137782364 ) ) ;
#117649=VERTEX_POINT ( 'NONE', #40857 ) ;
#117650=ORIENTED_EDGE ( 'NONE', *, *, #70820, .F. ) ;
#117651=VERTEX_POINT ( 'NONE', #71572 ) ;
#117652=ORIENTED_EDGE ( 'NONE', *, *, #8570, .T. ) ;
#117653=CARTESIAN_POINT ( 'NONE',  ( -5.600000000000020073, 12.50000000000000000, 3.918623584224383727 ) ) ;
#117654=FACE_BOUND ( 'NONE', #46436, .T. ) ;
#117655=VECTOR ( 'NONE', #120413, 1000.000000000000000 ) ;
#117656=AXIS2_PLACEMENT_3D ( 'NONE', #89586, #129539, #39865 ) ;
#117657=DIRECTION ( 'NONE',  ( 0.000000000000000000, 0.000000000000000000, 1.000000000000000000 ) ) ;
#117658=CONICAL_SURFACE ( 'NONE', #57039, 0.1000000000000000056, 0.003490658503988666988 ) ;
#117659=ORIENTED_EDGE ( 'NONE', *, *, #37984, .T. ) ;
#117660=FACE_OUTER_BOUND ( 'NONE', #38825, .T. ) ;
#117661=DIRECTION ( 'NONE',  ( 0.000000000000000000, -0.9999939076577903929, 0.003490651415223739937 ) ) ;
#117662=DIRECTION ( 'NONE',  ( 0.000000000000000000, 0.000000000000000000, -1.000000000000000000 ) ) ;
#117663=ORIENTED_EDGE ( 'NONE', *, *, #76212, .F. ) ;
#117664=AXIS2_PLACEMENT_3D ( 'NONE', #16218, #74528, #115724 ) ;
#117665=CARTESIAN_POINT ( 'NONE',  ( 6.849999999999929479, 12.50000000000000000, -2.446380397790840266 ) ) ;
#117666=DIRECTION ( 'NONE',  ( 0.000000000000000000, 1.000000000000000000, 0.000000000000000000 ) ) ;
#117667=EDGE_CURVE ( 'NONE', #49122, #62242, #80634, .T. ) ;
#117668=CONICAL_SURFACE ( 'NONE', #121805, 0.09999999999999999167, 0.003490658503988666988 ) ;
#117669=AXIS2_PLACEMENT_3D ( 'NONE', #29391, #9736, #32472 ) ;
#117670=EDGE_LOOP ( 'NONE', ( #34669, #21128, #5251, #33761 ) ) ;
#117671=EDGE_CURVE ( 'NONE', #128960, #113533, #53238, .T. ) ;
#117672=ORIENTED_EDGE ( 'NONE', *, *, #61887, .F. ) ;
#117673=EDGE_CURVE ( 'NONE', #65564, #123810, #36722, .T. ) ;
#117674=CARTESIAN_POINT ( 'NONE',  ( -2.300000000000033573, 2.500000000000000000, -4.083716857408426826 ) ) ;
#117675=DIRECTION ( 'NONE',  ( 0.000000000000000000, 1.000000000000000000, 0.000000000000000000 ) ) ;
#117676=VECTOR ( 'NONE', #21414, 1000.000000000000000 ) ;
#117677=ADVANCED_FACE ( 'NONE', ( #82031 ), #47180, .T. ) ;
#117678=EDGE_CURVE ( 'NONE', #52047, #76324, #22502, .T. ) ;
#117679=CARTESIAN_POINT ( 'NONE',  ( 4.149999999999938183, 2.500000000000000000, 7.088010851410848190 ) ) ;
#117680=DIRECTION ( 'NONE',  ( 0.000000000000000000, 0.000000000000000000, 1.000000000000000000 ) ) ;
#117681=ORIENTED_EDGE ( 'NONE', *, *, #82364, .T. ) ;
#117682=DIRECTION ( 'NONE',  ( 0.000000000000000000, 1.000000000000000000, 0.000000000000000000 ) ) ;
#117683=EDGE_CURVE ( 'NONE', #1124, #47988, #91081, .T. ) ;
#117684=VERTEX_POINT ( 'NONE', #3479 ) ;
#117685=ORIENTED_EDGE ( 'NONE', *, *, #117380, .T. ) ;
#117686=CARTESIAN_POINT ( 'NONE',  ( 3.749999999999940492, 2.500000000000000000, 5.802370205355744659 ) ) ;
#117687=ORIENTED_EDGE ( 'NONE', *, *, #98326, .T. ) ;
#117688=CARTESIAN_POINT ( 'NONE',  ( -3.350000000000032507, 12.50000000000000000, -6.495190528383302464 ) ) ;
#117689=FACE_BOUND ( 'NONE', #17852, .T. ) ;
#117690=EDGE_CURVE ( 'NONE', #52824, #98546, #34674, .T. ) ;
#117691=ADVANCED_FACE ( 'NONE', ( #126484 ), #53875, .T. ) ;
#117692=VERTEX_POINT ( 'NONE', #44703 ) ;
#117693=CARTESIAN_POINT ( 'NONE',  ( 2.899999999999946620, 12.50000000000000000, -3.572213422710612374 ) ) ;
#117694=ORIENTED_EDGE ( 'NONE', *, *, #113001, .F. ) ;
#117695=CARTESIAN_POINT ( 'NONE',  ( -10.85000000000000142, 2.500000000000000000, 6.495190528383297135 ) ) ;
#117696=DIRECTION ( 'NONE',  ( -0.000000000000000000, -1.000000000000000000, -0.000000000000000000 ) ) ;
#117697=DIRECTION ( 'NONE',  ( 0.000000000000000000, 1.000000000000000000, 0.000000000000000000 ) ) ;
#117698=CIRCLE ( 'NONE', #109406, 0.06509327318403743123 ) ;
#117699=CARTESIAN_POINT ( 'NONE',  ( 9.599999999999917932, 2.500000000000000000, -0.7928203230275542301 ) ) ;
#117700=CARTESIAN_POINT ( 'NONE',  ( 0.6499999999999566125, 12.50000000000000000, -6.083687093685488989 ) ) ;
#117701=ORIENTED_EDGE ( 'NONE', *, *, #52525, .F. ) ;
#117702=EDGE_LOOP ( 'NONE', ( #65050, #80908, #2445 ) ) ;
#117703=DIRECTION ( 'NONE',  ( 0.000000000000000000, 0.000000000000000000, 1.000000000000000000 ) ) ;
#117704=AXIS2_PLACEMENT_3D ( 'NONE', #115531, #35706, #43608 ) ;
#117705=AXIS2_PLACEMENT_3D ( 'NONE', #72620, #31411, #32064 ) ;
#117706=CARTESIAN_POINT ( 'NONE',  ( 0.5999999999999555689, 2.500000000000000000, 4.576537180435972019 ) ) ;
#117707=CONICAL_SURFACE ( 'NONE', #11104, 0.1000000000000002554, 0.003490658503988666988 ) ;
#117708=CONICAL_SURFACE ( 'NONE', #98849, 0.1000000000000002554, 0.003490658503988666988 ) ;
#117709=CARTESIAN_POINT ( 'NONE',  ( 6.049999999999930544, 2.500000000000000000, 2.611473670974873151 ) ) ;
#117710=ORIENTED_EDGE ( 'NONE', *, *, #90739, .T. ) ;
#117711=VERTEX_POINT ( 'NONE', #4744 ) ;
#117712=ORIENTED_EDGE ( 'NONE', *, *, #36885, .T. ) ;
#117713=CARTESIAN_POINT ( 'NONE',  ( 7.499999999999925393, 2.500000000000000000, 5.022947341949748790 ) ) ;
#117715=AXIS2_PLACEMENT_3D ( 'NONE', #58217, #107937, #68010 ) ;
#117716=CIRCLE ( 'NONE', #2710, 0.06509327318403745899 ) ;
#117717=AXIS2_PLACEMENT_3D ( 'NONE', #2185, #40863, #21857 ) ;
#117719=DIRECTION ( 'NONE',  ( -0.000000000000000000, -1.000000000000000000, -0.000000000000000000 ) ) ;
#117720=DIRECTION ( 'NONE',  ( 0.000000000000000000, -0.000000000000000000, 1.000000000000000000 ) ) ;
#117721=CARTESIAN_POINT ( 'NONE',  ( 6.849999999999929479, 12.50000000000000000, 6.841600689897072485 ) ) ;
#117722=CONICAL_SURFACE ( 'NONE', #17372, 0.1000000000000000472, 0.003490658503988666988 ) ;
#117723=CARTESIAN_POINT ( 'NONE',  ( 15.19999999999989093, 12.50000000000000000, 0.3464101615137735735 ) ) ;
#117724=CARTESIAN_POINT ( 'NONE',  ( 5.849999999999933920, 2.500000000000000000, 6.395190528383296602 ) ) ;
#117725=AXIS2_PLACEMENT_3D ( 'NONE', #114687, #75406, #23755 ) ;
#117727=AXIS2_PLACEMENT_3D ( 'NONE', #89120, #49220, #119866 ) ;
#117728=EDGE_LOOP ( 'NONE', ( #29365, #46724 ) ) ;
#117729=ORIENTED_EDGE ( 'NONE', *, *, #94997, .F. ) ;
#117730=DIRECTION ( 'NONE',  ( 0.000000000000000000, 1.000000000000000000, 0.000000000000000000 ) ) ;
#117731=DIRECTION ( 'NONE',  ( 0.000000000000000000, -0.000000000000000000, 1.000000000000000000 ) ) ;
#117732=VERTEX_POINT ( 'NONE', #44052 ) ;
#117733=VERTEX_POINT ( 'NONE', #125813 ) ;
#117735=DIRECTION ( 'NONE',  ( -0.000000000000000000, 1.000000000000000000, -0.000000000000000000 ) ) ;
#117736=DIRECTION ( 'NONE',  ( 0.000000000000000000, 0.000000000000000000, 1.000000000000000000 ) ) ;
#117738=EDGE_CURVE ( 'NONE', #54447, #22835, #112019, .T. ) ;
#117739=DIRECTION ( 'NONE',  ( -4.274815082592931898E-19, -0.9999939076577903929, -0.003490651415223739937 ) ) ;
#117740=DIRECTION ( 'NONE',  ( 0.000000000000000000, 1.000000000000000000, 0.000000000000000000 ) ) ;
#117741=DIRECTION ( 'NONE',  ( -0.000000000000000000, 1.000000000000000000, -0.000000000000000000 ) ) ;
#117742=ORIENTED_EDGE ( 'NONE', *, *, #105601, .T. ) ;
#117743=CARTESIAN_POINT ( 'NONE',  ( 8.549999999999920774, 12.50000000000000000, -2.511473670974877948 ) ) ;
#117744=VECTOR ( 'NONE', #86228, 1000.000000000000000 ) ;
#117745=DIRECTION ( 'NONE',  ( 0.000000000000000000, 0.000000000000000000, 1.000000000000000000 ) ) ;
#117746=CIRCLE ( 'NONE', #6924, 0.06509327318403745899 ) ;
#117747=AXIS2_PLACEMENT_3D ( 'NONE', #86077, #114906, #125391 ) ;
#117748=EDGE_LOOP ( 'NONE', ( #14414, #20151, #50074, #40126 ) ) ;
#117749=EDGE_LOOP ( 'NONE', ( #103885, #88191 ) ) ;
#117751=VERTEX_POINT ( 'NONE', #84623 ) ;
#117753=DIRECTION ( 'NONE',  ( -0.000000000000000000, -1.000000000000000000, -0.000000000000000000 ) ) ;
#117754=DIRECTION ( 'NONE',  ( -4.274815082592931898E-19, -0.9999939076577903929, -0.003490651415223739937 ) ) ;
#117755=CIRCLE ( 'NONE', #9008, 0.1000000000000002554 ) ;
#117756=CIRCLE ( 'NONE', #23695, 0.1000000000000000472 ) ;
#117757=ORIENTED_EDGE ( 'NONE', *, *, #111623, .T. ) ;
#117758=DIRECTION ( 'NONE',  ( 0.000000000000000000, 0.000000000000000000, -1.000000000000000000 ) ) ;
#117759=CARTESIAN_POINT ( 'NONE',  ( 17.50000000000000000, 0.9166666666666674068, -9.999999999999998224 ) ) ;
#117760=CARTESIAN_POINT ( 'NONE',  ( -2.050000000000033129, 2.500000000000000000, 6.495190528383297135 ) ) ;
#117761=DIRECTION ( 'NONE',  ( -0.000000000000000000, -1.000000000000000000, -0.000000000000000000 ) ) ;
#117762=ORIENTED_EDGE ( 'NONE', *, *, #96058, .T. ) ;
#117763=DIRECTION ( 'NONE',  ( 0.000000000000000000, 1.000000000000000000, 0.000000000000000000 ) ) ;
#117764=AXIS2_PLACEMENT_3D ( 'NONE', #90315, #123494, #33213 ) ;
#117765=FACE_OUTER_BOUND ( 'NONE', #79446, .T. ) ;
#117766=VERTEX_POINT ( 'NONE', #104261 ) ;
#117767=AXIS2_PLACEMENT_3D ( 'NONE', #37607, #129226, #68337 ) ;
#117768=AXIS2_PLACEMENT_3D ( 'NONE', #94701, #5023, #114975 ) ;
#117769=EDGE_LOOP ( 'NONE', ( #13877, #14030, #51077, #2288 ) ) ;
#117770=EDGE_LOOP ( 'NONE', ( #61556, #43038 ) ) ;
#117771=DIRECTION ( 'NONE',  ( 0.000000000000000000, 0.000000000000000000, -1.000000000000000000 ) ) ;
#117772=AXIS2_PLACEMENT_3D ( 'NONE', #120753, #112873, #61848 ) ;
#117774=VECTOR ( 'NONE', #106247, 1000.000000000000000 ) ;
#117775=EDGE_CURVE ( 'NONE', #79983, #83925, #13705, .T. ) ;
#117776=EDGE_LOOP ( 'NONE', ( #55755, #120168, #112296, #46936 ) ) ;
#117777=DIRECTION ( 'NONE',  ( 0.000000000000000000, 1.000000000000000000, 0.000000000000000000 ) ) ;
#117779=EDGE_CURVE ( 'NONE', #57084, #25471, #103624, .T. ) ;
#117780=DIRECTION ( 'NONE',  ( -0.000000000000000000, 1.000000000000000000, -0.000000000000000000 ) ) ;
#117781=DIRECTION ( 'NONE',  ( 0.000000000000000000, 0.000000000000000000, 1.000000000000000000 ) ) ;
#117782=EDGE_CURVE ( 'NONE', #102213, #104601, #3261, .T. ) ;
#117783=EDGE_LOOP ( 'NONE', ( #11116, #52424, #103939, #120446 ) ) ;
#117784=DIRECTION ( 'NONE',  ( 0.000000000000000000, 1.000000000000000000, 0.000000000000000000 ) ) ;
#117785=EDGE_LOOP ( 'NONE', ( #80960, #32148 ) ) ;
#117786=ADVANCED_FACE ( 'NONE', ( #85890 ), #76733, .T. ) ;
#117787=EDGE_CURVE ( 'NONE', #113497, #125598, #24411, .T. ) ;
#117788=EDGE_LOOP ( 'NONE', ( #67494, #101633, #88603, #35869 ) ) ;
#117789=CARTESIAN_POINT ( 'NONE',  ( -7.900000000000014566, 2.500000000000000000, -0.6928203230275541413 ) ) ;
#117791=AXIS2_PLACEMENT_3D ( 'NONE', #105315, #75205, #104648 ) ;
#117793=CARTESIAN_POINT ( 'NONE',  ( 2.049999999999950084, 12.50000000000000000, -6.495190528383302464 ) ) ;
#117794=EDGE_CURVE ( 'NONE', #90718, #89885, #30471, .T. ) ;
#117795=EDGE_CURVE ( 'NONE', #35451, #107061, #122398, .T. ) ;
#117796=FACE_BOUND ( 'NONE', #31384, .T. ) ;
#117797=DIRECTION ( 'NONE',  ( -0.000000000000000000, -1.000000000000000000, -0.000000000000000000 ) ) ;
#117798=CARTESIAN_POINT ( 'NONE',  ( 0.4499999999999569344, 2.500000000000000000, 2.265063509461097357 ) ) ;
#117799=CARTESIAN_POINT ( 'NONE',  ( 7.699999999999923794, 2.500000000000000000, -3.983716857408426293 ) ) ;
#117800=AXIS2_PLACEMENT_3D ( 'NONE', #101724, #82067, #108934 ) ;
#117801=AXIS2_PLACEMENT_3D ( 'NONE', #43103, #83015, #33276 ) ;
#117802=CONICAL_SURFACE ( 'NONE', #126144, 0.1000000000000002554, 0.003490658503988666988 ) ;
#117803=ORIENTED_EDGE ( 'NONE', *, *, #97582, .T. ) ;
#117806=ADVANCED_FACE ( 'NONE', ( #114717 ), #35535, .T. ) ;
#117807=DIRECTION ( 'NONE',  ( 0.000000000000000000, 0.000000000000000000, -1.000000000000000000 ) ) ;
#117808=CARTESIAN_POINT ( 'NONE',  ( 13.54999999999989946, 2.500000000000000000, 2.511473670974873507 ) ) ;
#117809=ORIENTED_EDGE ( 'NONE', *, *, #53279, .F. ) ;
#117810=CARTESIAN_POINT ( 'NONE',  ( 14.99999999999992895, 2.500000000000000000, -0.1000000000000022815 ) ) ;
#117811=AXIS2_PLACEMENT_3D ( 'NONE', #121920, #72190, #123217 ) ;
#117812=AXIS2_PLACEMENT_3D ( 'NONE', #1595, #13988, #81467 ) ;
#117813=CARTESIAN_POINT ( 'NONE',  ( -14.59999999999998366, 2.500000000000000000, 0.6928203230275518099 ) ) ;
#117814=EDGE_LOOP ( 'NONE', ( #27882, #101387, #7314, #64192 ) ) ;
#117815=ORIENTED_EDGE ( 'NONE', *, *, #39833, .T. ) ;
#117816=AXIS2_PLACEMENT_3D ( 'NONE', #51767, #10529, #21002 ) ;
#117817=DIRECTION ( 'NONE',  ( 0.000000000000000000, 1.000000000000000000, 0.000000000000000000 ) ) ;
#117818=DIRECTION ( 'NONE',  ( 0.000000000000000000, 1.000000000000000000, 0.000000000000000000 ) ) ;
#117819=FACE_BOUND ( 'NONE', #60997, .T. ) ;
#117820=CARTESIAN_POINT ( 'NONE',  ( 4.999999999999969802, 2.500000000000000000, 4.330127018922196314 ) ) ;
#117821=ORIENTED_EDGE ( 'NONE', *, *, #62769, .T. ) ;
#117822=LINE ( 'NONE', #127036, #52860 ) ;
#117823=EDGE_LOOP ( 'NONE', ( #102879, #62151 ) ) ;
#117825=ORIENTED_EDGE ( 'NONE', *, *, #89886, .F. ) ;
#117826=DIRECTION ( 'NONE',  ( 0.000000000000000000, 0.000000000000000000, 1.000000000000000000 ) ) ;
#117828=EDGE_LOOP ( 'NONE', ( #49415, #26466, #94623, #36723 ) ) ;
#117829=FACE_OUTER_BOUND ( 'NONE', #9294, .T. ) ;
#117830=DIRECTION ( 'NONE',  ( 0.000000000000000000, 0.000000000000000000, 1.000000000000000000 ) ) ;
#117831=EDGE_CURVE ( 'NONE', #9793, #45052, #65942, .T. ) ;
#117832=DIRECTION ( 'NONE',  ( 0.000000000000000000, 0.000000000000000000, -1.000000000000000000 ) ) ;
#117833=DIRECTION ( 'NONE',  ( 0.000000000000000000, -0.000000000000000000, 1.000000000000000000 ) ) ;
#117834=CIRCLE ( 'NONE', #61144, 0.06509327318403745899 ) ;
#117835=EDGE_CURVE ( 'NONE', #54631, #51919, #70165, .T. ) ;
#117836=VECTOR ( 'NONE', #22405, 1000.000000000000000 ) ;
#117837=ORIENTED_EDGE ( 'NONE', *, *, #31062, .F. ) ;
#117838=EDGE_CURVE ( 'NONE', #76450, #26951, #9522, .T. ) ;
#117839=DIRECTION ( 'NONE',  ( 0.000000000000000000, 1.000000000000000000, 0.000000000000000000 ) ) ;
#117840=LINE ( 'NONE', #127049, #112408 ) ;
#117841=DIRECTION ( 'NONE',  ( 0.000000000000000000, 0.000000000000000000, 1.000000000000000000 ) ) ;
#117842=FACE_OUTER_BOUND ( 'NONE', #49789, .T. ) ;
#117843=ORIENTED_EDGE ( 'NONE', *, *, #17486, .T. ) ;
#117844=DIRECTION ( 'NONE',  ( 0.000000000000000000, 1.000000000000000000, 0.000000000000000000 ) ) ;
#117845=VERTEX_POINT ( 'NONE', #4108 ) ;
#117846=ADVANCED_FACE ( 'NONE', ( #76091 ), #123884, .T. ) ;
#117847=CONICAL_SURFACE ( 'NONE', #19672, 0.09999999999999982514, 0.003490658503988666988 ) ;
#117848=CARTESIAN_POINT ( 'NONE',  ( 0.3999999999999563904, 2.500000000000000000, 3.637306695894644726 ) ) ;
#117849=VECTOR ( 'NONE', #8278, 1000.000000000000000 ) ;
#117850=EDGE_CURVE ( 'NONE', #32199, #11699, #86872, .T. ) ;
#117851=VERTEX_POINT ( 'NONE', #49871 ) ;
#117852=CONICAL_SURFACE ( 'NONE', #9202, 0.09999999999999982514, 0.003490658503988666988 ) ;
#117853=FACE_OUTER_BOUND ( 'NONE', #71031, .T. ) ;
#117854=DIRECTION ( 'NONE',  ( 0.000000000000000000, -0.000000000000000000, 1.000000000000000000 ) ) ;
#117855=EDGE_CURVE ( 'NONE', #57879, #62826, #45124, .T. ) ;
#117856=AXIS2_PLACEMENT_3D ( 'NONE', #36997, #17318, #17986 ) ;
#117857=DIRECTION ( 'NONE',  ( -0.000000000000000000, 1.000000000000000000, -0.000000000000000000 ) ) ;
#117858=ADVANCED_FACE ( 'NONE', ( #67530 ), #19075, .T. ) ;
#117859=FACE_OUTER_BOUND ( 'NONE', #75326, .T. ) ;
#117860=VERTEX_POINT ( 'NONE', #106818 ) ;
#117861=CARTESIAN_POINT ( 'NONE',  ( 6.249999999999932498, 12.50000000000000000, -2.857883832488653741 ) ) ;
#117862=DIRECTION ( 'NONE',  ( 0.000000000000000000, 1.000000000000000000, 0.000000000000000000 ) ) ;
#117863=CARTESIAN_POINT ( 'NONE',  ( -5.000000000000023093, 2.500000000000000000, 4.922947341949748257 ) ) ;
#117866=AXIS2_PLACEMENT_3D ( 'NONE', #17394, #46887, #126070 ) ;
#117868=EDGE_CURVE ( 'NONE', #3164, #2356, #63989, .T. ) ;
#117869=ORIENTED_EDGE ( 'NONE', *, *, #89790, .T. ) ;
#117870=ORIENTED_EDGE ( 'NONE', *, *, #5613, .F. ) ;
#117871=DIRECTION ( 'NONE',  ( 0.000000000000000000, -0.9999939076577903929, 0.003490651415223739937 ) ) ;
#117872=CIRCLE ( 'NONE', #82398, 0.06509327318403745899 ) ;
#117873=VERTEX_POINT ( 'NONE', #119231 ) ;
#117874=CIRCLE ( 'NONE', #105370, 0.06509327318403745899 ) ;
#117875=CIRCLE ( 'NONE', #11267, 0.06509327318403745899 ) ;
#117876=CARTESIAN_POINT ( 'NONE',  ( -2.500000000000030642, 2.500000000000000000, -0.6928203230275541413 ) ) ;
#117878=ORIENTED_EDGE ( 'NONE', *, *, #51059, .F. ) ;
#117879=VERTEX_POINT ( 'NONE', #98950 ) ;
#117880=CIRCLE ( 'NONE', #13417, 0.1000000000000002554 ) ;
#117881=DIRECTION ( 'NONE',  ( 0.000000000000000000, 1.000000000000000000, 0.000000000000000000 ) ) ;
#117882=AXIS2_PLACEMENT_3D ( 'NONE', #3689, #61981, #82909 ) ;
#117883=DIRECTION ( 'NONE',  ( -0.000000000000000000, -1.000000000000000000, -0.000000000000000000 ) ) ;
#117884=CARTESIAN_POINT ( 'NONE',  ( -13.34999999999999076, 12.50000000000000000, -2.857883832488651521 ) ) ;
#117885=DIRECTION ( 'NONE',  ( -0.000000000000000000, 1.000000000000000000, -0.000000000000000000 ) ) ;
#117886=CARTESIAN_POINT ( 'NONE',  ( 6.249999999999968914, 2.500000000000000000, -6.595190528383302109 ) ) ;
#117887=CARTESIAN_POINT ( 'NONE',  ( 6.449999999999931788, 12.50000000000000000, -6.148780366869526226 ) ) ;
#117888=DIRECTION ( 'NONE',  ( -4.274815082592931898E-19, -0.9999939076577903929, -0.003490651415223739937 ) ) ;
#117889=EDGE_CURVE ( 'NONE', #119822, #126385, #89034, .T. ) ;
#117890=DIRECTION ( 'NONE',  ( -0.000000000000000000, -1.000000000000000000, -0.000000000000000000 ) ) ;
#117891=ORIENTED_EDGE ( 'NONE', *, *, #119037, .F. ) ;
#117892=ORIENTED_EDGE ( 'NONE', *, *, #126105, .F. ) ;
#117893=ORIENTED_EDGE ( 'NONE', *, *, #52619, .T. ) ;
#117894=ORIENTED_EDGE ( 'NONE', *, *, #103334, .F. ) ;
#117895=AXIS2_PLACEMENT_3D ( 'NONE', #110824, #92480, #61094 ) ;
#117896=DIRECTION ( 'NONE',  ( 0.000000000000000000, 1.000000000000000000, 0.000000000000000000 ) ) ;
#117897=AXIS2_PLACEMENT_3D ( 'NONE', #54791, #35812, #84908 ) ;
#117898=AXIS2_PLACEMENT_3D ( 'NONE', #90825, #31914, #90154 ) ;
#117899=ORIENTED_EDGE ( 'NONE', *, *, #66827, .F. ) ;
#117900=EDGE_LOOP ( 'NONE', ( #71854, #106480, #31217, #17228 ) ) ;
#117901=AXIS2_PLACEMENT_3D ( 'NONE', #44740, #125223, #93830 ) ;
#117902=CARTESIAN_POINT ( 'NONE',  ( -13.54999999999999005, 2.500000000000000000, 2.511473670974877503 ) ) ;
#117903=AXIS2_PLACEMENT_3D ( 'NONE', #101841, #60009, #90067 ) ;
#117904=CARTESIAN_POINT ( 'NONE',  ( -8.750000000000010658, 2.500000000000000000, 2.857883832488649301 ) ) ;
#117905=ADVANCED_FACE ( 'NONE', ( #47283 ), #124631, .T. ) ;
#117906=AXIS2_PLACEMENT_3D ( 'NONE', #8789, #79491, #97821 ) ;
#117907=DIRECTION ( 'NONE',  ( 0.000000000000000000, 1.000000000000000000, 0.000000000000000000 ) ) ;
#117908=CARTESIAN_POINT ( 'NONE',  ( 3.749999999999978684, 12.50000000000000000, -6.495190528383302464 ) ) ;
#117909=CONICAL_SURFACE ( 'NONE', #82335, 0.1000000000000002554, 0.003490658503988666988 ) ;
#117910=CARTESIAN_POINT ( 'NONE',  ( 6.449999999999930012, 12.50000000000000000, -1.818653347947326138 ) ) ;
#117911=ORIENTED_EDGE ( 'NONE', *, *, #84455, .T. ) ;
#117912=FACE_OUTER_BOUND ( 'NONE', #49016, .T. ) ;
#117913=CONICAL_SURFACE ( 'NONE', #42644, 0.1000000000000002554, 0.003490658503988666988 ) ;
#117914=CIRCLE ( 'NONE', #63555, 0.1000000000000000472 ) ;
#117915=ORIENTED_EDGE ( 'NONE', *, *, #37576, .F. ) ;
#117916=DIRECTION ( 'NONE',  ( 0.000000000000000000, 0.000000000000000000, -1.000000000000000000 ) ) ;
#117917=AXIS2_PLACEMENT_3D ( 'NONE', #109314, #19657, #27515 ) ;
#117918=ORIENTED_EDGE ( 'NONE', *, *, #122287, .T. ) ;
#117919=DIRECTION ( 'NONE',  ( -0.000000000000000000, -1.000000000000000000, -0.000000000000000000 ) ) ;
#117920=VERTEX_POINT ( 'NONE', #128436 ) ;
#117921=CIRCLE ( 'NONE', #860, 0.06509327318403745899 ) ;
#117922=EDGE_CURVE ( 'NONE', #63043, #107053, #7536, .T. ) ;
#117923=ORIENTED_EDGE ( 'NONE', *, *, #26089, .F. ) ;
#117924=DIRECTION ( 'NONE',  ( -0.000000000000000000, 1.000000000000000000, -0.000000000000000000 ) ) ;
#117925=CARTESIAN_POINT ( 'NONE',  ( 87.50000000000001421, -3.975350567648449740, -6.360562287258772152 ) ) ;
#117926=DIRECTION ( 'NONE',  ( 0.000000000000000000, 1.000000000000000000, 0.000000000000000000 ) ) ;
#117927=FACE_OUTER_BOUND ( 'NONE', #64630, .T. ) ;
#117928=AXIS2_PLACEMENT_3D ( 'NONE', #110805, #72194, #32284 ) ;
#117929=CARTESIAN_POINT ( 'NONE',  ( -1.450000000000036371, 2.500000000000000000, 6.841600689897072485 ) ) ;
#117930=ORIENTED_EDGE ( 'NONE', *, *, #102303, .T. ) ;
#117931=DIRECTION ( 'NONE',  ( -0.000000000000000000, 1.000000000000000000, -0.000000000000000000 ) ) ;
#117933=CARTESIAN_POINT ( 'NONE',  ( -9.150000000000009237, 2.500000000000000000, -7.288010851410849256 ) ) ;
#117934=DIRECTION ( 'NONE',  ( 0.000000000000000000, 1.000000000000000000, 0.000000000000000000 ) ) ;
#117935=AXIS2_PLACEMENT_3D ( 'NONE', #126133, #86186, #48221 ) ;
#117936=CARTESIAN_POINT ( 'NONE',  ( 10.39999999999991154, 2.500000000000000000, 3.637306695894644726 ) ) ;
#117937=VERTEX_POINT ( 'NONE', #26997 ) ;
#117938=VERTEX_POINT ( 'NONE', #7979 ) ;
#117939=DIRECTION ( 'NONE',  ( 0.000000000000000000, 0.000000000000000000, -1.000000000000000000 ) ) ;
#117940=ORIENTED_EDGE ( 'NONE', *, *, #762, .F. ) ;
#117941=AXIS2_PLACEMENT_3D ( 'NONE', #62010, #31900, #84201 ) ;
#117942=DIRECTION ( 'NONE',  ( -0.000000000000000000, -1.000000000000000000, -0.000000000000000000 ) ) ;
#117943=CARTESIAN_POINT ( 'NONE',  ( -14.19999999999998685, 12.50000000000000000, -1.084202172485504434E-16 ) ) ;
#117944=ADVANCED_FACE ( 'NONE', ( #66898 ), #116201, .T. ) ;
#117945=VERTEX_POINT ( 'NONE', #7332 ) ;
#117947=CARTESIAN_POINT ( 'NONE',  ( -6.250000000000015987, 2.500000000000000000, 5.802370205355744659 ) ) ;
#117948=CARTESIAN_POINT ( 'NONE',  ( -3.550000000000028244, 12.50000000000000000, -1.818653347947326138 ) ) ;
#117949=DIRECTION ( 'NONE',  ( 0.000000000000000000, 0.000000000000000000, 1.000000000000000000 ) ) ;
#117950=EDGE_LOOP ( 'NONE', ( #95007, #99718, #33617, #114496 ) ) ;
#117951=EDGE_CURVE ( 'NONE', #66296, #6219, #86967, .T. ) ;
#117952=AXIS2_PLACEMENT_3D ( 'NONE', #100422, #10721, #50672 ) ;
#117953=DIRECTION ( 'NONE',  ( 0.000000000000000000, 1.000000000000000000, 0.000000000000000000 ) ) ;
#117954=CARTESIAN_POINT ( 'NONE',  ( -13.09999999999999076, 2.500000000000000000, 3.983716857408420964 ) ) ;
#117955=VERTEX_POINT ( 'NONE', #57082 ) ;
#117956=EDGE_CURVE ( 'NONE', #79243, #109920, #18004, .T. ) ;
#117957=ADVANCED_FACE ( 'NONE', ( #117266 ), #91182, .T. ) ;
#117958=EDGE_CURVE ( 'NONE', #20142, #80050, #49350, .T. ) ;
#117959=DIRECTION ( 'NONE',  ( 0.000000000000000000, 0.000000000000000000, 1.000000000000000000 ) ) ;
#117960=EDGE_CURVE ( 'NONE', #64674, #10550, #49228, .T. ) ;
#117961=FACE_OUTER_BOUND ( 'NONE', #60875, .T. ) ;
#117962=DIRECTION ( 'NONE',  ( 0.000000000000000000, 0.000000000000000000, 1.000000000000000000 ) ) ;
#117963=ORIENTED_EDGE ( 'NONE', *, *, #116802, .T. ) ;
#117964=CIRCLE ( 'NONE', #17617, 0.09999999999999982514 ) ;
#117965=VECTOR ( 'NONE', #91109, 1000.000000000000000 ) ;
#117966=DIRECTION ( 'NONE',  ( 0.000000000000000000, -0.9999939076577903929, 0.003490651415223739937 ) ) ;
#117967=CIRCLE ( 'NONE', #51104, 0.09999999999999982514 ) ;
#117969=FACE_OUTER_BOUND ( 'NONE', #46734, .T. ) ;
#117970=CARTESIAN_POINT ( 'NONE',  ( -4.293440603042597559E-14, 2.500000000000000000, 5.122947341949749323 ) ) ;
#117971=EDGE_CURVE ( 'NONE', #55580, #88783, #8609, .T. ) ;
#117972=DIRECTION ( 'NONE',  ( 0.000000000000000000, 0.000000000000000000, -1.000000000000000000 ) ) ;
#117973=AXIS2_PLACEMENT_3D ( 'NONE', #29151, #58603, #117474 ) ;
#117974=ORIENTED_EDGE ( 'NONE', *, *, #19389, .T. ) ;
#117975=EDGE_CURVE ( 'NONE', #10181, #87020, #72320, .T. ) ;
#117976=CARTESIAN_POINT ( 'NONE',  ( -2.100000000000034284, 2.500000000000000000, -4.230127018922201998 ) ) ;
#117977=EDGE_CURVE ( 'NONE', #66966, #81045, #107894, .T. ) ;
#117978=FACE_OUTER_BOUND ( 'NONE', #64758, .T. ) ;
#117979=ORIENTED_EDGE ( 'NONE', *, *, #11329, .T. ) ;
#117980=CARTESIAN_POINT ( 'NONE',  ( -0.4000000000000404898, 2.500000000000000000, 5.022947341949748790 ) ) ;
#117981=VERTEX_POINT ( 'NONE', #69475 ) ;
#117982=DIRECTION ( 'NONE',  ( 0.000000000000000000, 0.000000000000000000, 1.000000000000000000 ) ) ;
#117983=VECTOR ( 'NONE', #30848, 1000.000000000000000 ) ;
#117984=EDGE_LOOP ( 'NONE', ( #106435, #87450, #112136, #116279 ) ) ;
#117985=CYLINDRICAL_SURFACE ( 'NONE', #6570, 1.000000000000000888 ) ;
#117986=CARTESIAN_POINT ( 'NONE',  ( 11.64999999999990798, 2.500000000000000000, -2.857883832488653741 ) ) ;
#117987=AXIS2_PLACEMENT_3D ( 'NONE', #27587, #77997, #58377 ) ;
#117988=VECTOR ( 'NONE', #123386, 1000.000000000000000 ) ;
#117989=ORIENTED_EDGE ( 'NONE', *, *, #33174, .T. ) ;
#117990=ORIENTED_EDGE ( 'NONE', *, *, #21054, .T. ) ;
#117991=FACE_OUTER_BOUND ( 'NONE', #97371, .T. ) ;
#117992=DIRECTION ( 'NONE',  ( 0.000000000000000000, 1.000000000000000000, 0.000000000000000000 ) ) ;
#117993=ORIENTED_EDGE ( 'NONE', *, *, #75095, .F. ) ;
#117994=CARTESIAN_POINT ( 'NONE',  ( 11.64999999999990266, 12.50000000000000000, 2.230156782645134950 ) ) ;
#117996=CIRCLE ( 'NONE', #122221, 0.1000000000000002554 ) ;
#117997=AXIS2_PLACEMENT_3D ( 'NONE', #27536, #85187, #15135 ) ;
#117998=CONICAL_SURFACE ( 'NONE', #61595, 0.1000000000000002554, 0.003490658503988666988 ) ;
#117999=DIRECTION ( 'NONE',  ( -4.274815082592931898E-19, -0.9999939076577903929, -0.003490651415223739937 ) ) ;
#118000=DIRECTION ( 'NONE',  ( 0.000000000000000000, 1.000000000000000000, 0.000000000000000000 ) ) ;
#118001=VECTOR ( 'NONE', #26188, 1000.000000000000000 ) ;
#118002=DIRECTION ( 'NONE',  ( 0.000000000000000000, -0.9999939076577903929, 0.003490651415223739937 ) ) ;
#118003=CARTESIAN_POINT ( 'NONE',  ( 12.69999999999990159, 2.500000000000000000, 4.676537180435972552 ) ) ;
#118004=AXIS2_PLACEMENT_3D ( 'NONE', #65427, #94247, #84431 ) ;
#118005=CIRCLE ( 'NONE', #30302, 0.06509327318403745899 ) ;
#118006=EDGE_LOOP ( 'NONE', ( #126453, #101517, #17090, #53338 ) ) ;
#118007=ORIENTED_EDGE ( 'NONE', *, *, #65516, .T. ) ;
#118009=ORIENTED_EDGE ( 'NONE', *, *, #18073, .F. ) ;
#118010=DIRECTION ( 'NONE',  ( -0.000000000000000000, -1.000000000000000000, -0.000000000000000000 ) ) ;
#118012=AXIS2_PLACEMENT_3D ( 'NONE', #113758, #54812, #14240 ) ;
#118013=CARTESIAN_POINT ( 'NONE',  ( 9.149999999999916866, 12.50000000000000000, -1.472243186433550122 ) ) ;
#118014=ORIENTED_EDGE ( 'NONE', *, *, #33434, .T. ) ;
#118015=FACE_BOUND ( 'NONE', #33022, .T. ) ;
#118016=ORIENTED_EDGE ( 'NONE', *, *, #99457, .T. ) ;
#118017=EDGE_CURVE ( 'NONE', #63986, #98143, #126685, .T. ) ;
#118018=CARTESIAN_POINT ( 'NONE',  ( -14.99999999999998401, 12.50000000000000000, 0.7579135962115892688 ) ) ;
#118019=LINE ( 'NONE', #46710, #75156 ) ;
#118020=ADVANCED_FACE ( 'NONE', ( #81249 ), #51152, .T. ) ;
#118021=DIRECTION ( 'NONE',  ( 0.000000000000000000, 1.000000000000000000, 0.000000000000000000 ) ) ;
#118022=FACE_OUTER_BOUND ( 'NONE', #63369, .T. ) ;
#118023=EDGE_CURVE ( 'NONE', #65136, #97390, #57742, .T. ) ;
#118024=DIRECTION ( 'NONE',  ( -0.000000000000000000, 1.000000000000000000, -0.000000000000000000 ) ) ;
#118025=DIRECTION ( 'NONE',  ( 0.000000000000000000, 0.000000000000000000, -1.000000000000000000 ) ) ;
#118026=PLANE ( 'NONE',  #81271 ) ;
#118027=DIRECTION ( 'NONE',  ( -0.000000000000000000, -1.000000000000000000, -0.000000000000000000 ) ) ;
#118028=CARTESIAN_POINT ( 'NONE',  ( 10.84999999999991260, 2.500000000000000000, -2.857883832488653741 ) ) ;
#118029=LINE ( 'NONE', #68279, #127505 ) ;
#118030=ADVANCED_FACE ( 'NONE', ( #91061 ), #62260, .T. ) ;
#118031=ORIENTED_EDGE ( 'NONE', *, *, #92835, .T. ) ;
#118033=ORIENTED_EDGE ( 'NONE', *, *, #10766, .F. ) ;
#118034=VERTEX_POINT ( 'NONE', #61617 ) ;
#118035=CARTESIAN_POINT ( 'NONE',  ( 16.64732342996689596, -0.5906619305413305376, -5.996708608239496030 ) ) ;
#118036=CARTESIAN_POINT ( 'NONE',  ( -7.950000000000012612, 2.500000000000000000, 2.165063509461097713 ) ) ;
#118037=ORIENTED_EDGE ( 'NONE', *, *, #16582, .F. ) ;
#118038=EDGE_LOOP ( 'NONE', ( #61820, #2490, #31328, #10021 ) ) ;
#118039=VERTEX_POINT ( 'NONE', #22973 ) ;
#118040=CARTESIAN_POINT ( 'NONE',  ( 2.099999999999950351, 12.50000000000000000, -4.265033745738164406 ) ) ;
#118041=AXIS2_PLACEMENT_3D ( 'NONE', #105132, #104493, #95964 ) ;
#118042=CIRCLE ( 'NONE', #118131, 0.1000000000000002554 ) ;
#118043=CARTESIAN_POINT ( 'NONE',  ( 0.4499999999999569344, 12.50000000000000000, -2.099970236277064473 ) ) ;
#118044=DIRECTION ( 'NONE',  ( -0.000000000000000000, 1.000000000000000000, -0.000000000000000000 ) ) ;
#118045=CARTESIAN_POINT ( 'NONE',  ( 1.849999999999950573, 2.500000000000000000, 2.411473670974873862 ) ) ;
#118046=DIRECTION ( 'NONE',  ( 0.000000000000000000, 0.000000000000000000, -1.000000000000000000 ) ) ;
#118047=CARTESIAN_POINT ( 'NONE',  ( 6.249999999999965361, 12.50000000000000000, 2.165063509461097713 ) ) ;
#118048=DIRECTION ( 'NONE',  ( 0.000000000000000000, 1.000000000000000000, 0.000000000000000000 ) ) ;
#118049=EDGE_CURVE ( 'NONE', #87436, #11640, #82790, .T. ) ;
#118050=VERTEX_POINT ( 'NONE', #13121 ) ;
#118051=DIRECTION ( 'NONE',  ( 0.000000000000000000, 1.000000000000000000, 0.000000000000000000 ) ) ;
#118052=VERTEX_POINT ( 'NONE', #11199 ) ;
#118053=CIRCLE ( 'NONE', #61634, 0.1000000000000002554 ) ;
#118054=ORIENTED_EDGE ( 'NONE', *, *, #78360, .T. ) ;
#118055=ORIENTED_EDGE ( 'NONE', *, *, #32351, .F. ) ;
#118056=AXIS2_PLACEMENT_3D ( 'NONE', #74704, #16397, #44602 ) ;
#118057=CARTESIAN_POINT ( 'NONE',  ( -2.700000000000029932, 2.500000000000000000, -4.676537180435977881 ) ) ;
#118058=VERTEX_POINT ( 'NONE', #112642 ) ;
#118059=ORIENTED_EDGE ( 'NONE', *, *, #43160, .T. ) ;
#118060=DIRECTION ( 'NONE',  ( -4.274815082592931898E-19, -0.9999939076577903929, -0.003490651415223739937 ) ) ;
#118061=DIRECTION ( 'NONE',  ( 0.000000000000000000, 0.000000000000000000, -1.000000000000000000 ) ) ;
#118062=CIRCLE ( 'NONE', #3061, 0.06509327318403745899 ) ;
#118063=LINE ( 'NONE', #125941, #83367 ) ;
#118064=CIRCLE ( 'NONE', #95092, 0.06509327318403745899 ) ;
#118065=ADVANCED_FACE ( 'NONE', ( #60949 ), #121164, .T. ) ;
#118066=DIRECTION ( 'NONE',  ( -0.000000000000000000, 1.000000000000000000, -0.000000000000000000 ) ) ;
#118067=CARTESIAN_POINT ( 'NONE',  ( -1.450000000000035483, 2.500000000000000000, 6.048780366869521252 ) ) ;
#118068=AXIS2_PLACEMENT_3D ( 'NONE', #10477, #22750, #3725 ) ;
#118069=VERTEX_POINT ( 'NONE', #1381 ) ;
#118070=CIRCLE ( 'NONE', #30269, 0.06509327318403745899 ) ;
#118071=CARTESIAN_POINT ( 'NONE',  ( -9.150000000000009237, 2.500000000000000000, -2.957883832488653830 ) ) ;
#118072=VERTEX_POINT ( 'NONE', #100867 ) ;
#118073=CARTESIAN_POINT ( 'NONE',  ( 21.25104878432635758, 0.2455272941110370200, 4.189300629079955485 ) ) ;
#118074=EDGE_LOOP ( 'NONE', ( #17780, #119260 ) ) ;
#118075=CARTESIAN_POINT ( 'NONE',  ( -13.94999999999998685, 12.50000000000000000, -2.511473670974875727 ) ) ;
#118076=DIRECTION ( 'NONE',  ( 0.000000000000000000, 1.000000000000000000, 0.000000000000000000 ) ) ;
#118077=ORIENTED_EDGE ( 'NONE', *, *, #70273, .F. ) ;
#118078=CARTESIAN_POINT ( 'NONE',  ( -5.850000000000019185, 2.500000000000000000, 2.165063509461097713 ) ) ;
#118079=ADVANCED_FACE ( 'NONE', ( #53074 ), #11754, .T. ) ;
#118080=CARTESIAN_POINT ( 'NONE',  ( 0.3999999999999559464, 2.500000000000000000, -4.230127018922201998 ) ) ;
#118081=EDGE_LOOP ( 'NONE', ( #113206, #50845 ) ) ;
#118082=CIRCLE ( 'NONE', #5202, 0.09999999999999982514 ) ;
#118083=CARTESIAN_POINT ( 'NONE',  ( 1.249999999999953815, 12.50000000000000000, -2.792790559304616504 ) ) ;
#118084=ORIENTED_EDGE ( 'NONE', *, *, #89318, .F. ) ;
#118085=AXIS2_PLACEMENT_3D ( 'NONE', #48174, #97269, #38373 ) ;
#118086=EDGE_CURVE ( 'NONE', #21308, #114987, #47276, .T. ) ;
#118087=ORIENTED_EDGE ( 'NONE', *, *, #112201, .T. ) ;
#118088=DIRECTION ( 'NONE',  ( 0.000000000000000000, 1.000000000000000000, 0.000000000000000000 ) ) ;
#118089=CARTESIAN_POINT ( 'NONE',  ( 13.09999999999990195, 2.500000000000000000, -4.083716857408426826 ) ) ;
#118091=CARTESIAN_POINT ( 'NONE',  ( -11.24999999999999822, 2.500000000000000000, 5.802370205355744659 ) ) ;
#118092=AXIS2_PLACEMENT_3D ( 'NONE', #58036, #121297, #72211 ) ;
#118093=DIRECTION ( 'NONE',  ( -0.000000000000000000, 1.000000000000000000, -0.000000000000000000 ) ) ;
#118094=CIRCLE ( 'NONE', #111849, 0.09999999999999982514 ) ;
#118095=DIRECTION ( 'NONE',  ( -0.000000000000000000, -1.000000000000000000, -0.000000000000000000 ) ) ;
#118096=AXIS2_PLACEMENT_3D ( 'NONE', #21359, #69821, #101216 ) ;
#118097=ORIENTED_EDGE ( 'NONE', *, *, #5381, .T. ) ;
#118099=DIRECTION ( 'NONE',  ( 0.000000000000000000, 1.000000000000000000, 0.000000000000000000 ) ) ;
#118100=DIRECTION ( 'NONE',  ( -4.274815082592931898E-19, -0.9999939076577903929, -0.003490651415223739937 ) ) ;
#118101=AXIS2_PLACEMENT_3D ( 'NONE', #32413, #93241, #94510 ) ;
#118102=EDGE_CURVE ( 'NONE', #104178, #31905, #2024, .T. ) ;
#118103=EDGE_LOOP ( 'NONE', ( #54232, #102986 ) ) ;
#118104=AXIS2_PLACEMENT_3D ( 'NONE', #68835, #9277, #17119 ) ;
#118105=CARTESIAN_POINT ( 'NONE',  ( 2.899999999999946620, 2.500000000000000000, 0.6928203230275494784 ) ) ;
#118106=DIRECTION ( 'NONE',  ( -0.000000000000000000, -1.000000000000000000, -0.000000000000000000 ) ) ;
#118107=DIRECTION ( 'NONE',  ( 0.000000000000000000, 1.000000000000000000, 0.000000000000000000 ) ) ;
#118108=CARTESIAN_POINT ( 'NONE',  ( -12.09999999999999609, 2.500000000000000000, 4.230127018922196669 ) ) ;
#118109=DIRECTION ( 'NONE',  ( 0.000000000000000000, 0.000000000000000000, -1.000000000000000000 ) ) ;
#118111=EDGE_CURVE ( 'NONE', #82534, #23974, #128767, .T. ) ;
#118112=CARTESIAN_POINT ( 'NONE',  ( 8.149999999999923972, 12.50000000000000000, 1.818653347947321475 ) ) ;
#118113=CARTESIAN_POINT ( 'NONE',  ( 8.349999999999919709, 12.50000000000000000, -2.165063509461101710 ) ) ;
#118114=EDGE_CURVE ( 'NONE', #115792, #21808, #38982, .T. ) ;
#118115=EDGE_CURVE ( 'NONE', #64039, #129191, #121800, .T. ) ;
#118116=EDGE_CURVE ( 'NONE', #87809, #83720, #118357, .T. ) ;
#118117=ADVANCED_FACE ( 'NONE', ( #119876 ), #30232, .T. ) ;
#118118=CIRCLE ( 'NONE', #15704, 0.1000000000000002554 ) ;
#118120=LINE ( 'NONE', #28469, #72007 ) ;
#118121=VERTEX_POINT ( 'NONE', #122468 ) ;
#118122=VERTEX_POINT ( 'NONE', #32806 ) ;
#118124=EDGE_CURVE ( 'NONE', #96385, #66216, #61942, .T. ) ;
#118125=EDGE_CURVE ( 'NONE', #46700, #89750, #737, .T. ) ;
#118126=ORIENTED_EDGE ( 'NONE', *, *, #108634, .T. ) ;
#118127=FACE_OUTER_BOUND ( 'NONE', #526, .T. ) ;
#118128=CARTESIAN_POINT ( 'NONE',  ( 11.89999999999990443, 2.500000000000000000, -0.2464101615137782308 ) ) ;
#118129=EDGE_CURVE ( 'NONE', #127931, #100949, #66102, .T. ) ;
#118130=CARTESIAN_POINT ( 'NONE',  ( 9.599999999999914380, 2.500000000000000000, -3.637306695894650055 ) ) ;
#118131=AXIS2_PLACEMENT_3D ( 'NONE', #37196, #124281, #34627 ) ;
#118132=VERTEX_POINT ( 'NONE', #25522 ) ;
#118133=ADVANCED_FACE ( 'NONE', ( #43908 ), #45215, .T. ) ;
#118134=CARTESIAN_POINT ( 'NONE',  ( 7.499999999999925393, 12.50000000000000000, -0.7579135962115916003 ) ) ;
#118135=EDGE_CURVE ( 'NONE', #8551, #27240, #53709, .T. ) ;
#118136=FACE_OUTER_BOUND ( 'NONE', #103675, .T. ) ;
#118137=ORIENTED_EDGE ( 'NONE', *, *, #18417, .T. ) ;
#118138=FACE_OUTER_BOUND ( 'NONE', #98407, .T. ) ;
#118139=EDGE_CURVE ( 'NONE', #43500, #53553, #41026, .T. ) ;
#118140=CARTESIAN_POINT ( 'NONE',  ( -9.150000000000009237, 2.500000000000000000, -2.857883832488653741 ) ) ;
#118141=ADVANCED_FACE ( 'NONE', ( #63540 ), #26191, .T. ) ;
#118142=VERTEX_POINT ( 'NONE', #64814 ) ;
#118143=AXIS2_PLACEMENT_3D ( 'NONE', #36040, #15736, #106696 ) ;
#118144=EDGE_LOOP ( 'NONE', ( #31863, #91671 ) ) ;
#118145=AXIS2_PLACEMENT_3D ( 'NONE', #78444, #58150, #39805 ) ;
#118146=ORIENTED_EDGE ( 'NONE', *, *, #115858, .F. ) ;
#118147=DIRECTION ( 'NONE',  ( -4.274815082592931898E-19, -0.9999939076577903929, -0.003490651415223739937 ) ) ;
#118148=DIRECTION ( 'NONE',  ( -0.000000000000000000, -1.000000000000000000, -0.000000000000000000 ) ) ;
#118149=DIRECTION ( 'NONE',  ( -0.000000000000000000, -1.000000000000000000, -0.000000000000000000 ) ) ;
#118150=FACE_BOUND ( 'NONE', #12646, .T. ) ;
#118151=ORIENTED_EDGE ( 'NONE', *, *, #63455, .F. ) ;
#118152=DIRECTION ( 'NONE',  ( 0.000000000000000000, 0.000000000000000000, -1.000000000000000000 ) ) ;
#118153=CARTESIAN_POINT ( 'NONE',  ( -2.900000000000030553, 2.500000000000000000, 4.922947341949748257 ) ) ;
#118155=DIRECTION ( 'NONE',  ( 0.000000000000000000, -0.9999939076577903929, 0.003490651415223739937 ) ) ;
#118156=VECTOR ( 'NONE', #100453, 1000.000000000000000 ) ;
#118157=DIRECTION ( 'NONE',  ( -0.000000000000000000, -1.000000000000000000, -0.000000000000000000 ) ) ;
#118158=CONICAL_SURFACE ( 'NONE', #9501, 0.1000000000000002554, 0.003490658503988666988 ) ;
#118159=DIRECTION ( 'NONE',  ( 0.000000000000000000, -0.9999939076577903929, 0.003490651415223739937 ) ) ;
#118160=DIRECTION ( 'NONE',  ( -0.000000000000000000, 1.000000000000000000, -0.000000000000000000 ) ) ;
#118161=DIRECTION ( 'NONE',  ( 0.000000000000000000, 0.000000000000000000, -1.000000000000000000 ) ) ;
#118162=DIRECTION ( 'NONE',  ( 0.000000000000000000, -0.000000000000000000, 1.000000000000000000 ) ) ;
#118163=CARTESIAN_POINT ( 'NONE',  ( 6.049999999999932321, 2.500000000000000000, 1.818653347947321475 ) ) ;
#118164=ORIENTED_EDGE ( 'NONE', *, *, #65682, .T. ) ;
#118165=ORIENTED_EDGE ( 'NONE', *, *, #42302, .T. ) ;
#118166=ORIENTED_EDGE ( 'NONE', *, *, #58146, .T. ) ;
#118167=AXIS2_PLACEMENT_3D ( 'NONE', #1168, #90169, #69916 ) ;
#118168=ORIENTED_EDGE ( 'NONE', *, *, #8937, .T. ) ;
#118169=VERTEX_POINT ( 'NONE', #13777 ) ;
#118170=CARTESIAN_POINT ( 'NONE',  ( -2.950000000000029932, 12.50000000000000000, -2.230156782645139391 ) ) ;
#118171=CARTESIAN_POINT ( 'NONE',  ( -8.749999999999975131, 12.50000000000000000, -2.165063509461101710 ) ) ;
#118173=FACE_BOUND ( 'NONE', #121904, .T. ) ;
#118174=AXIS2_PLACEMENT_3D ( 'NONE', #124353, #123062, #33408 ) ;
#118175=DIRECTION ( 'NONE',  ( 0.000000000000000000, 0.000000000000000000, -1.000000000000000000 ) ) ;
#118176=ADVANCED_FACE ( 'NONE', ( #125027 ), #95472, .T. ) ;
#118177=AXIS2_PLACEMENT_3D ( 'NONE', #103928, #82371, #22169 ) ;
#118178=DIRECTION ( 'NONE',  ( 0.000000000000000000, 0.000000000000000000, 1.000000000000000000 ) ) ;
#118179=AXIS2_PLACEMENT_3D ( 'NONE', #27145, #95886, #55949 ) ;
#118180=EDGE_CURVE ( 'NONE', #56415, #123846, #95384, .T. ) ;
#118181=AXIS2_PLACEMENT_3D ( 'NONE', #7272, #77315, #54448 ) ;
#118183=CARTESIAN_POINT ( 'NONE',  ( -6.071532165918824830E-15, 2.500000000000000000, -4.230127018922201998 ) ) ;
#118184=PLANE ( 'NONE',  #114476 ) ;
#118185=EDGE_LOOP ( 'NONE', ( #47734, #87876 ) ) ;
#118186=CARTESIAN_POINT ( 'NONE',  ( 11.64999999999990798, 12.50000000000000000, -2.857883832488653741 ) ) ;
#118187=AXIS2_PLACEMENT_3D ( 'NONE', #64935, #14546, #95711 ) ;
#118188=EDGE_CURVE ( 'NONE', #10182, #112593, #72501, .T. ) ;
#118189=VERTEX_POINT ( 'NONE', #14416 ) ;
#118190=CIRCLE ( 'NONE', #78508, 0.06509327318403745899 ) ;
#118191=CONICAL_SURFACE ( 'NONE', #49254, 0.1000000000000002554, 0.003490658503988666988 ) ;
#118192=EDGE_LOOP ( 'NONE', ( #60521, #91912, #34441, #29115 ) ) ;
#118193=ORIENTED_EDGE ( 'NONE', *, *, #11631, .T. ) ;
#118194=DIRECTION ( 'NONE',  ( -0.000000000000000000, -1.000000000000000000, -0.000000000000000000 ) ) ;
#118195=AXIS2_PLACEMENT_3D ( 'NONE', #113607, #114886, #114250 ) ;
#118196=CARTESIAN_POINT ( 'NONE',  ( 6.598553918464142853, 2.500000000000000000, 8.770211965307137092 ) ) ;
#118197=CARTESIAN_POINT ( 'NONE',  ( 0.6499999999999561684, 2.500000000000000000, 1.818653347947321475 ) ) ;
#118198=ORIENTED_EDGE ( 'NONE', *, *, #91798, .T. ) ;
#118199=FACE_OUTER_BOUND ( 'NONE', #123392, .T. ) ;
#118200=AXIS2_PLACEMENT_3D ( 'NONE', #73426, #81333, #12570 ) ;
#118201=DIRECTION ( 'NONE',  ( -0.000000000000000000, 1.000000000000000000, -0.000000000000000000 ) ) ;
#118202=AXIS2_PLACEMENT_3D ( 'NONE', #95045, #13885, #92452 ) ;
#118203=DIRECTION ( 'NONE',  ( 0.000000000000000000, -0.000000000000000000, 1.000000000000000000 ) ) ;
#118205=CARTESIAN_POINT ( 'NONE',  ( 6.849999999999929479, 12.50000000000000000, -1.818653347947326138 ) ) ;
#118206=CARTESIAN_POINT ( 'NONE',  ( -12.69999999999999218, 2.500000000000000000, 4.576537180435972019 ) ) ;
#118207=CIRCLE ( 'NONE', #76442, 0.1000000000000002554 ) ;
#118208=FACE_OUTER_BOUND ( 'NONE', #106722, .T. ) ;
#118209=VERTEX_POINT ( 'NONE', #104103 ) ;
#118210=FACE_OUTER_BOUND ( 'NONE', #42736, .T. ) ;
#118211=ORIENTED_EDGE ( 'NONE', *, *, #105284, .T. ) ;
#118212=VERTEX_POINT ( 'NONE', #83186 ) ;
#118213=CARTESIAN_POINT ( 'NONE',  ( 6.049999999999932321, 2.500000000000000000, 6.841600689897072485 ) ) ;
#118214=DIRECTION ( 'NONE',  ( 0.000000000000000000, 0.000000000000000000, 1.000000000000000000 ) ) ;
#118215=CARTESIAN_POINT ( 'NONE',  ( -11.64999999999999680, 2.500000000000000000, 5.802370205355744659 ) ) ;
#118216=AXIS2_PLACEMENT_3D ( 'NONE', #75348, #5956, #116562 ) ;
#118217=ORIENTED_EDGE ( 'NONE', *, *, #26962, .T. ) ;
#118218=ORIENTED_EDGE ( 'NONE', *, *, #48127, .F. ) ;
#118219=EDGE_CURVE ( 'NONE', #115955, #22580, #75923, .T. ) ;
#118220=DIRECTION ( 'NONE',  ( 0.000000000000000000, 1.000000000000000000, 0.000000000000000000 ) ) ;
#118221=DIRECTION ( 'NONE',  ( -0.000000000000000000, 1.000000000000000000, -0.000000000000000000 ) ) ;
#118222=CARTESIAN_POINT ( 'NONE',  ( -15.39999999999997904, 2.500000000000000000, 0.000000000000000000 ) ) ;
#118223=VERTEX_POINT ( 'NONE', #36013 ) ;
#118224=VERTEX_POINT ( 'NONE', #93642 ) ;
#118225=CARTESIAN_POINT ( 'NONE',  ( -6.249999999999981348, 2.500000000000000000, 2.265063509461097357 ) ) ;
#118226=AXIS2_PLACEMENT_3D ( 'NONE', #50564, #61701, #120604 ) ;
#118227=ADVANCED_FACE ( 'NONE', ( #123103 ), #68273, .T. ) ;
#118228=AXIS2_PLACEMENT_3D ( 'NONE', #19843, #7420, #68927 ) ;
#118229=ORIENTED_EDGE ( 'NONE', *, *, #101596, .T. ) ;
#118230=CARTESIAN_POINT ( 'NONE',  ( 7.099999999999928590, 2.500000000000000000, 3.637306695894644726 ) ) ;
#118231=DIRECTION ( 'NONE',  ( -0.000000000000000000, 1.000000000000000000, -0.000000000000000000 ) ) ;
#118232=ORIENTED_EDGE ( 'NONE', *, *, #52950, .T. ) ;
#118233=DIRECTION ( 'NONE',  ( 0.000000000000000000, 0.000000000000000000, 1.000000000000000000 ) ) ;
#118234=FACE_OUTER_BOUND ( 'NONE', #50537, .T. ) ;
#118235=DIRECTION ( 'NONE',  ( -0.000000000000000000, 1.000000000000000000, -0.000000000000000000 ) ) ;
#118236=EDGE_CURVE ( 'NONE', #91313, #11053, #105394, .T. ) ;
#118237=EDGE_CURVE ( 'NONE', #65076, #106610, #80813, .T. ) ;
#118238=PLANE ( 'NONE',  #41670 ) ;
#118239=ORIENTED_EDGE ( 'NONE', *, *, #74835, .F. ) ;
#118240=CONICAL_SURFACE ( 'NONE', #49314, 0.09999999999999999167, 0.003490658503988666988 ) ;
#118241=DIRECTION ( 'NONE',  ( 0.000000000000000000, 0.000000000000000000, 1.000000000000000000 ) ) ;
#118242=EDGE_LOOP ( 'NONE', ( #54036, #117681, #35926, #35011 ) ) ;
#118243=ORIENTED_EDGE ( 'NONE', *, *, #78244, .F. ) ;
#118244=EDGE_CURVE ( 'NONE', #3245, #27692, #54352, .T. ) ;
#118245=CARTESIAN_POINT ( 'NONE',  ( -4.600000000000028066, 12.50000000000000000, -3.702399969078687292 ) ) ;
#118246=CARTESIAN_POINT ( 'NONE',  ( 11.44999999999991047, 2.500000000000000000, 6.148780366869520009 ) ) ;
#118247=CARTESIAN_POINT ( 'NONE',  ( -0.6500000000000403233, 12.50000000000000000, 1.883746621131358934 ) ) ;
#118248=DIRECTION ( 'NONE',  ( -0.000000000000000000, -1.000000000000000000, -0.000000000000000000 ) ) ;
#118249=CARTESIAN_POINT ( 'NONE',  ( -5.450000000000019718, 2.500000000000000000, 2.165063509461097713 ) ) ;
#118250=CARTESIAN_POINT ( 'NONE',  ( 6.899999999999928413, 12.50000000000000000, -4.048810130592463530 ) ) ;
#118251=AXIS2_PLACEMENT_3D ( 'NONE', #69539, #107544, #110120 ) ;
#118252=AXIS2_PLACEMENT_3D ( 'NONE', #74085, #26282, #35462 ) ;
#118253=PLANE ( 'NONE',  #92689 ) ;
#118254=LINE ( 'NONE', #60010, #59564 ) ;
#118255=LINE ( 'NONE', #30548, #88090 ) ;
#118256=LINE ( 'NONE', #77675, #89835 ) ;
#118257=ORIENTED_EDGE ( 'NONE', *, *, #97552, .F. ) ;
#118258=PLANE ( 'NONE',  #127879 ) ;
#118259=CARTESIAN_POINT ( 'NONE',  ( 4.149999999999941735, 12.50000000000000000, -7.188010851410854052 ) ) ;
#118260=DIRECTION ( 'NONE',  ( 0.000000000000000000, 0.000000000000000000, -1.000000000000000000 ) ) ;
#118261=CARTESIAN_POINT ( 'NONE',  ( -2.050000000000033129, 2.500000000000000000, 2.165063509461097713 ) ) ;
#118262=FACE_OUTER_BOUND ( 'NONE', #70345, .T. ) ;
#118263=ORIENTED_EDGE ( 'NONE', *, *, #103554, .T. ) ;
#118264=DIRECTION ( 'NONE',  ( 0.000000000000000000, 1.000000000000000000, 0.000000000000000000 ) ) ;
#118265=EDGE_CURVE ( 'NONE', #91647, #77185, #74000, .T. ) ;
#118266=AXIS2_PLACEMENT_3D ( 'NONE', #34897, #6041, #64336 ) ;
#118267=CARTESIAN_POINT ( 'NONE',  ( -1.850000000000033396, 2.500000000000000000, -2.511473670974877948 ) ) ;
#118268=LINE ( 'NONE', #8306, #115238 ) ;
#118269=ORIENTED_EDGE ( 'NONE', *, *, #101586, .F. ) ;
#118270=ADVANCED_FACE ( 'NONE', ( #34743 ), #4576, .T. ) ;
#118271=EDGE_CURVE ( 'NONE', #73967, #39963, #122581, .T. ) ;
#118272=ORIENTED_EDGE ( 'NONE', *, *, #99345, .T. ) ;
#118273=DIRECTION ( 'NONE',  ( 0.000000000000000000, 0.000000000000000000, 1.000000000000000000 ) ) ;
#118274=VERTEX_POINT ( 'NONE', #106670 ) ;
#118275=VERTEX_POINT ( 'NONE', #79173 ) ;
#118277=DIRECTION ( 'NONE',  ( 0.000000000000000000, 0.000000000000000000, 1.000000000000000000 ) ) ;
#118278=EDGE_CURVE ( 'NONE', #87285, #77424, #87033, .T. ) ;
#118279=CIRCLE ( 'NONE', #5409, 0.1000000000000002554 ) ;
#118281=EDGE_CURVE ( 'NONE', #98563, #119463, #126782, .T. ) ;
#118282=LINE ( 'NONE', #67892, #94580 ) ;
#118283=CARTESIAN_POINT ( 'NONE',  ( -13.94999999999998863, 12.50000000000000000, 2.511473670974877503 ) ) ;
#118284=AXIS2_PLACEMENT_3D ( 'NONE', #61773, #10691, #30382 ) ;
#118285=DIRECTION ( 'NONE',  ( -4.274815082592931898E-19, -0.9999939076577903929, -0.003490651415223739937 ) ) ;
#118286=AXIS2_PLACEMENT_3D ( 'NONE', #52349, #111920, #73276 ) ;
#118287=ORIENTED_EDGE ( 'NONE', *, *, #64657, .T. ) ;
#118288=AXIS2_PLACEMENT_3D ( 'NONE', #25640, #127087, #56389 ) ;
#118289=EDGE_CURVE ( 'NONE', #81973, #49584, #1371, .T. ) ;
#118290=CARTESIAN_POINT ( 'NONE',  ( -3.750000000000031086, 2.500000000000000000, -5.902370205355750521 ) ) ;
#118291=AXIS2_PLACEMENT_3D ( 'NONE', #100709, #91550, #121642 ) ;
#118292=ORIENTED_EDGE ( 'NONE', *, *, #55971, .T. ) ;
#118293=DIRECTION ( 'NONE',  ( 0.000000000000000000, 0.000000000000000000, -1.000000000000000000 ) ) ;
#118294=CARTESIAN_POINT ( 'NONE',  ( 15.44463772191480899, -2.469073678227705848, -4.264595835270768909 ) ) ;
#118295=CARTESIAN_POINT ( 'NONE',  ( 17.88933034088993068, 0.4802206367765988193, 4.999988745079567920 ) ) ;
#118296=CARTESIAN_POINT ( 'NONE',  ( 10.59999999999990905, 12.50000000000000000, -3.983716857408426293 ) ) ;
#118297=CARTESIAN_POINT ( 'NONE',  ( -12.09999999999999609, 2.500000000000000000, -4.330127018922198978 ) ) ;
#118298=ADVANCED_FACE ( 'NONE', ( #56912 ), #18101, .T. ) ;
#118299=ORIENTED_EDGE ( 'NONE', *, *, #19990, .F. ) ;
#118300=ORIENTED_EDGE ( 'NONE', *, *, #98613, .T. ) ;
#118301=ORIENTED_EDGE ( 'NONE', *, *, #2274, .T. ) ;
#118302=ORIENTED_EDGE ( 'NONE', *, *, #4265, .T. ) ;
#118303=ORIENTED_EDGE ( 'NONE', *, *, #90621, .F. ) ;
#118304=CARTESIAN_POINT ( 'NONE',  ( 12.49999999999993960, 2.500000000000000000, -4.230127018922201998 ) ) ;
#118305=CARTESIAN_POINT ( 'NONE',  ( -6.650000000000014566, 12.50000000000000000, 5.802370205355744659 ) ) ;
#118306=CARTESIAN_POINT ( 'NONE',  ( 0.1999999999999562961, 12.50000000000000000, 4.676537180435972552 ) ) ;
#118307=FACE_BOUND ( 'NONE', #22981, .T. ) ;
#118308=DIRECTION ( 'NONE',  ( 0.000000000000000000, 0.000000000000000000, -1.000000000000000000 ) ) ;
#118309=VECTOR ( 'NONE', #24821, 1000.000000000000000 ) ;
#118310=DIRECTION ( 'NONE',  ( -4.274815082592931898E-19, -0.9999939076577903929, -0.003490651415223739937 ) ) ;
#118311=DIRECTION ( 'NONE',  ( -0.000000000000000000, -1.000000000000000000, -0.000000000000000000 ) ) ;
#118312=CARTESIAN_POINT ( 'NONE',  ( -0.6500000000000394351, 2.500000000000000000, 6.741600689897071952 ) ) ;
#118314=AXIS2_PLACEMENT_3D ( 'NONE', #102098, #62188, #100169 ) ;
#118315=CARTESIAN_POINT ( 'NONE',  ( -4.150000000000024336, 12.50000000000000000, -2.165063509461101710 ) ) ;
#118316=CARTESIAN_POINT ( 'NONE',  ( -8.100000000000013856, 2.500000000000000000, 0.4464101615137736623 ) ) ;
#118317=AXIS2_PLACEMENT_3D ( 'NONE', #122041, #32395, #36239 ) ;
#118318=AXIS2_PLACEMENT_3D ( 'NONE', #101103, #103027, #83410 ) ;
#118319=CARTESIAN_POINT ( 'NONE',  ( 1.849999999999950573, 12.50000000000000000, 2.511473670974873507 ) ) ;
#118321=ORIENTED_EDGE ( 'NONE', *, *, #85311, .T. ) ;
#118322=VERTEX_POINT ( 'NONE', #87671 ) ;
#118323=ORIENTED_EDGE ( 'NONE', *, *, #50320, .T. ) ;
#118324=ORIENTED_EDGE ( 'NONE', *, *, #45859, .T. ) ;
#118325=DIRECTION ( 'NONE',  ( 0.000000000000000000, 0.000000000000000000, -1.000000000000000000 ) ) ;
#118326=DIRECTION ( 'NONE',  ( 0.000000000000000000, -0.9999939076577903929, 0.003490651415223739937 ) ) ;
#118327=FACE_BOUND ( 'NONE', #37386, .T. ) ;
#118328=AXIS2_PLACEMENT_3D ( 'NONE', #35887, #75795, #115723 ) ;
#118329=DIRECTION ( 'NONE',  ( 0.000000000000000000, -0.9999939076577903929, 0.003490651415223739937 ) ) ;
#118330=ADVANCED_FACE ( 'NONE', ( #86385 ), #15940, .T. ) ;
#118331=CIRCLE ( 'NONE', #22213, 0.1000000000000002554 ) ;
#118332=CIRCLE ( 'NONE', #32593, 0.06509327318403745899 ) ;
#118333=VERTEX_POINT ( 'NONE', #38609 ) ;
#118334=DIRECTION ( 'NONE',  ( 0.000000000000000000, 0.000000000000000000, -1.000000000000000000 ) ) ;
#118335=DIRECTION ( 'NONE',  ( -0.000000000000000000, -1.000000000000000000, -0.000000000000000000 ) ) ;
#118336=DIRECTION ( 'NONE',  ( 0.000000000000000000, 0.000000000000000000, 1.000000000000000000 ) ) ;
#118337=DIRECTION ( 'NONE',  ( -4.274815082592931898E-19, -0.9999939076577903929, -0.003490651415223739937 ) ) ;
#118338=ORIENTED_EDGE ( 'NONE', *, *, #52100, .T. ) ;
#118339=DIRECTION ( 'NONE',  ( -0.000000000000000000, 1.000000000000000000, -0.000000000000000000 ) ) ;
#118340=ADVANCED_FACE ( 'NONE', ( #36670 ), #67361, .T. ) ;
#118341=ORIENTED_EDGE ( 'NONE', *, *, #115906, .F. ) ;
#118342=ORIENTED_EDGE ( 'NONE', *, *, #25155, .T. ) ;
#118343=FACE_OUTER_BOUND ( 'NONE', #12769, .T. ) ;
#118344=CARTESIAN_POINT ( 'NONE',  ( 0.6499999999999561684, 2.500000000000000000, 1.918653347947321564 ) ) ;
#118345=ORIENTED_EDGE ( 'NONE', *, *, #84847, .F. ) ;
#118346=DIRECTION ( 'NONE',  ( 0.000000000000000000, 1.000000000000000000, 0.000000000000000000 ) ) ;
#118347=DIRECTION ( 'NONE',  ( -0.000000000000000000, 1.000000000000000000, -0.000000000000000000 ) ) ;
#118348=ORIENTED_EDGE ( 'NONE', *, *, #88179, .F. ) ;
#118349=CARTESIAN_POINT ( 'NONE',  ( -9.550000000000002487, 12.50000000000000000, 6.430097255199259010 ) ) ;
#118350=ORIENTED_EDGE ( 'NONE', *, *, #81365, .F. ) ;
#118351=CARTESIAN_POINT ( 'NONE',  ( -12.49999999999999289, 2.500000000000000000, -0.6928203230275500335 ) ) ;
#118352=EDGE_LOOP ( 'NONE', ( #61105, #42706, #13204, #98696 ) ) ;
#118354=FACE_BOUND ( 'NONE', #45242, .T. ) ;
#118355=VECTOR ( 'NONE', #106759, 1000.000000000000000 ) ;
#118356=ORIENTED_EDGE ( 'NONE', *, *, #113232, .T. ) ;
#118357=CIRCLE ( 'NONE', #99506, 0.06509327318403745899 ) ;
#118359=EDGE_LOOP ( 'NONE', ( #30972, #61620, #47719, #108705 ) ) ;
#118360=CARTESIAN_POINT ( 'NONE',  ( -7.499999999999980460, 12.50000000000000000, -0.06509327318403970719 ) ) ;
#118361=DIRECTION ( 'NONE',  ( 0.000000000000000000, 0.000000000000000000, -1.000000000000000000 ) ) ;
#118362=CARTESIAN_POINT ( 'NONE',  ( 4.349999999999938360, 12.50000000000000000, 1.818653347947321475 ) ) ;
#118363=CARTESIAN_POINT ( 'NONE',  ( -6.900000000000015454, 2.500000000000000000, 3.883716857408420431 ) ) ;
#118364=DIRECTION ( 'NONE',  ( 0.000000000000000000, 0.000000000000000000, 1.000000000000000000 ) ) ;
#118365=VERTEX_POINT ( 'NONE', #116487 ) ;
#118366=VECTOR ( 'NONE', #56796, 1000.000000000000000 ) ;
#118367=ORIENTED_EDGE ( 'NONE', *, *, #95818, .F. ) ;
#118368=EDGE_CURVE ( 'NONE', #79214, #51306, #120519, .T. ) ;
#118369=ORIENTED_EDGE ( 'NONE', *, *, #19328, .F. ) ;
#118370=DIRECTION ( 'NONE',  ( 0.000000000000000000, 1.000000000000000000, 0.000000000000000000 ) ) ;
#118371=CARTESIAN_POINT ( 'NONE',  ( 6.249999999999934275, 2.500000000000000000, -7.188010851410854052 ) ) ;
#118372=DIRECTION ( 'NONE',  ( 0.000000000000000000, 1.000000000000000000, 0.000000000000000000 ) ) ;
#118373=ORIENTED_EDGE ( 'NONE', *, *, #74389, .F. ) ;
#118374=ORIENTED_EDGE ( 'NONE', *, *, #99654, .T. ) ;
#118375=VERTEX_POINT ( 'NONE', #109245 ) ;
#118376=CARTESIAN_POINT ( 'NONE',  ( 0.8499999999999550138, 12.50000000000000000, -5.867463478539787225 ) ) ;
#118377=AXIS2_PLACEMENT_3D ( 'NONE', #66896, #36172, #108115 ) ;
#118378=DIRECTION ( 'NONE',  ( 0.000000000000000000, 1.000000000000000000, 0.000000000000000000 ) ) ;
#118379=EDGE_CURVE ( 'NONE', #65189, #103138, #77852, .T. ) ;
#118380=CIRCLE ( 'NONE', #72425, 0.09999999999999982514 ) ;
#118381=FACE_OUTER_BOUND ( 'NONE', #14494, .T. ) ;
#118382=PLANE ( 'NONE',  #89928 ) ;
#118383=DIRECTION ( 'NONE',  ( 0.000000000000000000, 0.000000000000000000, -1.000000000000000000 ) ) ;
#118384=DIRECTION ( 'NONE',  ( 0.000000000000000000, 1.000000000000000000, 0.000000000000000000 ) ) ;
#118385=CARTESIAN_POINT ( 'NONE',  ( 4.149999999999941735, 12.50000000000000000, -5.802370205355749988 ) ) ;
#118386=EDGE_CURVE ( 'NONE', #61065, #5316, #16032, .T. ) ;
#118387=EDGE_CURVE ( 'NONE', #91313, #79119, #64080, .T. ) ;
#118388=PLANE ( 'NONE',  #75006 ) ;
#118390=VERTEX_POINT ( 'NONE', #39260 ) ;
#118391=LINE ( 'NONE', #119049, #63306 ) ;
#118392=EDGE_CURVE ( 'NONE', #57054, #119412, #76598, .T. ) ;
#118394=ORIENTED_EDGE ( 'NONE', *, *, #66103, .T. ) ;
#118395=VERTEX_POINT ( 'NONE', #28128 ) ;
#118396=EDGE_CURVE ( 'NONE', #3681, #48754, #107971, .T. ) ;
#118398=CARTESIAN_POINT ( 'NONE',  ( -10.85000000000000142, 12.50000000000000000, 6.495190528383297135 ) ) ;
#118399=VECTOR ( 'NONE', #61379, 1000.000000000000000 ) ;
#118400=DIRECTION ( 'NONE',  ( -0.000000000000000000, 1.000000000000000000, -0.000000000000000000 ) ) ;
#118401=DIRECTION ( 'NONE',  ( 0.000000000000000000, 1.000000000000000000, 0.000000000000000000 ) ) ;
#118402=DIRECTION ( 'NONE',  ( 0.000000000000000000, 1.000000000000000000, 0.000000000000000000 ) ) ;
#118403=CIRCLE ( 'NONE', #66166, 0.09999999999999999167 ) ;
#118404=AXIS2_PLACEMENT_3D ( 'NONE', #45493, #97156, #46119 ) ;
#118405=CARTESIAN_POINT ( 'NONE',  ( 4.349999999999939249, 2.500000000000000000, 2.511473670974873507 ) ) ;
#118406=CARTESIAN_POINT ( 'NONE',  ( 0.1999999999999562961, 12.50000000000000000, 4.676537180435972552 ) ) ;
#118407=CIRCLE ( 'NONE', #68224, 0.09999999999999982514 ) ;
#118408=VECTOR ( 'NONE', #22089, 1000.000000000000000 ) ;
#118409=CIRCLE ( 'NONE', #61990, 0.09999999999999982514 ) ;
#118410=DIRECTION ( 'NONE',  ( 0.000000000000000000, 0.000000000000000000, 1.000000000000000000 ) ) ;
#118411=ORIENTED_EDGE ( 'NONE', *, *, #70838, .F. ) ;
#118412=CIRCLE ( 'NONE', #93377, 0.1000000000000002554 ) ;
#118413=EDGE_LOOP ( 'NONE', ( #80304, #40803, #69763, #16909 ) ) ;
#118414=ORIENTED_EDGE ( 'NONE', *, *, #70690, .F. ) ;
#118415=ORIENTED_EDGE ( 'NONE', *, *, #749, .T. ) ;
#118416=DIRECTION ( 'NONE',  ( -0.000000000000000000, 1.000000000000000000, -0.000000000000000000 ) ) ;
#118417=DIRECTION ( 'NONE',  ( 0.000000000000000000, 0.000000000000000000, 1.000000000000000000 ) ) ;
#118418=AXIS2_PLACEMENT_3D ( 'NONE', #47978, #8655, #36865 ) ;
#118419=ORIENTED_EDGE ( 'NONE', *, *, #101435, .T. ) ;
#118420=CARTESIAN_POINT ( 'NONE',  ( -10.65000000000000391, 2.500000000000000000, -2.511473670974873951 ) ) ;
#118421=ADVANCED_FACE ( 'NONE', ( #8460 ), #89121, .T. ) ;
#118422=FACE_OUTER_BOUND ( 'NONE', #43877, .T. ) ;
#118423=CIRCLE ( 'NONE', #78737, 0.09999999999999982514 ) ;
#118424=DIRECTION ( 'NONE',  ( 0.000000000000000000, 0.000000000000000000, 1.000000000000000000 ) ) ;
#118425=CARTESIAN_POINT ( 'NONE',  ( -3.750000000000025757, 2.500000000000000000, -2.957883832488653830 ) ) ;
#118426=EDGE_LOOP ( 'NONE', ( #72963, #22413, #2666, #106804 ) ) ;
#118428=EDGE_CURVE ( 'NONE', #109103, #54777, #99597, .T. ) ;
#118429=CARTESIAN_POINT ( 'NONE',  ( 9.599999999999914380, 2.500000000000000000, 5.022947341949748790 ) ) ;
#118430=ORIENTED_EDGE ( 'NONE', *, *, #74984, .T. ) ;
#118431=VERTEX_POINT ( 'NONE', #108609 ) ;
#118432=ORIENTED_EDGE ( 'NONE', *, *, #14187, .T. ) ;
#118433=DIRECTION ( 'NONE',  ( 0.000000000000000000, -0.000000000000000000, 1.000000000000000000 ) ) ;
#118434=EDGE_CURVE ( 'NONE', #86996, #80440, #82874, .T. ) ;
#118435=EDGE_CURVE ( 'NONE', #72665, #2195, #87051, .T. ) ;
#118436=EDGE_CURVE ( 'NONE', #87633, #63269, #32712, .T. ) ;
#118437=DIRECTION ( 'NONE',  ( -0.000000000000000000, 1.000000000000000000, -0.000000000000000000 ) ) ;
#118438=EDGE_CURVE ( 'NONE', #17267, #98189, #124716, .T. ) ;
#118439=EDGE_LOOP ( 'NONE', ( #104573, #28880, #57017, #11771 ) ) ;
#118440=DIRECTION ( 'NONE',  ( 0.000000000000000000, -0.9999939076577903929, 0.003490651415223739937 ) ) ;
#118441=CARTESIAN_POINT ( 'NONE',  ( -12.29999999999999716, 2.500000000000000000, 0.3464101615137776813 ) ) ;
#118442=LINE ( 'NONE', #108624, #108940 ) ;
#118443=CARTESIAN_POINT ( 'NONE',  ( 6.649999999999931077, 2.500000000000000000, -6.495190528383302464 ) ) ;
#118444=ADVANCED_FACE ( 'NONE', ( #101379 ), #11836, .T. ) ;
#118445=ORIENTED_EDGE ( 'NONE', *, *, #10809, .F. ) ;
#118446=EDGE_CURVE ( 'NONE', #33924, #36661, #41191, .T. ) ;
#118447=CIRCLE ( 'NONE', #95471, 0.06509327318403745899 ) ;
#118448=DIRECTION ( 'NONE',  ( 0.000000000000000000, 0.000000000000000000, -1.000000000000000000 ) ) ;
#118449=EDGE_LOOP ( 'NONE', ( #27615, #2394, #40482, #104931 ) ) ;
#118451=CARTESIAN_POINT ( 'NONE',  ( -0.4000000000000392131, 12.50000000000000000, -4.265033745738164406 ) ) ;
#118452=CARTESIAN_POINT ( 'NONE',  ( 12.29999999999990301, 12.50000000000000000, -0.3464101615137782364 ) ) ;
#118453=FACE_BOUND ( 'NONE', #9417, .T. ) ;
#118454=DIRECTION ( 'NONE',  ( 0.000000000000000000, -0.000000000000000000, 1.000000000000000000 ) ) ;
#118455=DIRECTION ( 'NONE',  ( 0.000000000000000000, 1.000000000000000000, 0.000000000000000000 ) ) ;
#118456=AXIS2_PLACEMENT_3D ( 'NONE', #45206, #15052, #24265 ) ;
#118457=VECTOR ( 'NONE', #29620, 1000.000000000000000 ) ;
#118458=DIRECTION ( 'NONE',  ( -0.000000000000000000, 1.000000000000000000, -0.000000000000000000 ) ) ;
#118459=VERTEX_POINT ( 'NONE', #12336 ) ;
#118460=DIRECTION ( 'NONE',  ( 0.000000000000000000, 0.000000000000000000, -1.000000000000000000 ) ) ;
#118461=FACE_OUTER_BOUND ( 'NONE', #104592, .T. ) ;
#118462=CONICAL_SURFACE ( 'NONE', #55779, 0.09999999999999982514, 0.003490658503988666988 ) ;
#118463=FACE_OUTER_BOUND ( 'NONE', #123991, .T. ) ;
#118464=DIRECTION ( 'NONE',  ( 0.000000000000000000, 0.000000000000000000, 1.000000000000000000 ) ) ;
#118465=ORIENTED_EDGE ( 'NONE', *, *, #34042, .F. ) ;
#118466=CIRCLE ( 'NONE', #5581, 0.09999999999999982514 ) ;
#118467=CARTESIAN_POINT ( 'NONE',  ( -7.900000000000014566, 2.500000000000000000, -4.430127018922202176 ) ) ;
#118468=AXIS2_PLACEMENT_3D ( 'NONE', #6737, #129157, #36892 ) ;
#118469=DIRECTION ( 'NONE',  ( 0.000000000000000000, 0.000000000000000000, -1.000000000000000000 ) ) ;
#118470=ORIENTED_EDGE ( 'NONE', *, *, #120807, .T. ) ;
#118471=ORIENTED_EDGE ( 'NONE', *, *, #27899, .F. ) ;
#118472=PLANE ( 'NONE',  #14638 ) ;
#118473=CARTESIAN_POINT ( 'NONE',  ( -10.65000000000000391, 12.50000000000000000, -2.511473670974873951 ) ) ;
#118474=FACE_BOUND ( 'NONE', #53356, .T. ) ;
#118475=CARTESIAN_POINT ( 'NONE',  ( 14.69205215198098102, -2.499999999999999112, -6.336420067969235959 ) ) ;
#118476=ORIENTED_EDGE ( 'NONE', *, *, #39230, .F. ) ;
#118477=FACE_OUTER_BOUND ( 'NONE', #69826, .T. ) ;
#118478=ORIENTED_EDGE ( 'NONE', *, *, #86, .F. ) ;
#118479=ORIENTED_EDGE ( 'NONE', *, *, #70316, .T. ) ;
#118480=DIRECTION ( 'NONE',  ( -4.274815082592931898E-19, -0.9999939076577903929, -0.003490651415223739937 ) ) ;
#118482=CONICAL_SURFACE ( 'NONE', #1696, 0.1000000000000002554, 0.003490658503988666988 ) ;
#118483=EDGE_LOOP ( 'NONE', ( #127237, #83665 ) ) ;
#118484=DIRECTION ( 'NONE',  ( -0.000000000000000000, 1.000000000000000000, -0.000000000000000000 ) ) ;
#118485=CONICAL_SURFACE ( 'NONE', #62080, 0.1000000000000002554, 0.003490658503988666988 ) ;
#118486=CARTESIAN_POINT ( 'NONE',  ( 9.399999999999915090, 2.500000000000000000, 3.983716857408420964 ) ) ;
#118487=ADVANCED_FACE ( 'NONE', ( #70621 ), #57828, .T. ) ;
#118488=CIRCLE ( 'NONE', #95519, 0.09999999999999999167 ) ;
#118489=DIRECTION ( 'NONE',  ( 0.000000000000000000, -0.000000000000000000, 1.000000000000000000 ) ) ;
#118490=DIRECTION ( 'NONE',  ( 0.000000000000000000, 1.000000000000000000, 0.000000000000000000 ) ) ;
#118491=CIRCLE ( 'NONE', #3487, 0.09999999999999982514 ) ;
#118492=AXIS2_PLACEMENT_3D ( 'NONE', #9017, #31265, #48974 ) ;
#118493=ORIENTED_EDGE ( 'NONE', *, *, #74247, .F. ) ;
#118496=DIRECTION ( 'NONE',  ( -4.274815082592931898E-19, -0.9999939076577903929, -0.003490651415223739937 ) ) ;
#118497=DIRECTION ( 'NONE',  ( -0.000000000000000000, 1.000000000000000000, -0.000000000000000000 ) ) ;
#118498=CARTESIAN_POINT ( 'NONE',  ( -7.900000000000014566, 12.50000000000000000, 0.7579135962115869374 ) ) ;
#118499=ORIENTED_EDGE ( 'NONE', *, *, #40631, .T. ) ;
#118500=CARTESIAN_POINT ( 'NONE',  ( -1.450000000000035039, 12.50000000000000000, -2.576566944158915184 ) ) ;
#118501=EDGE_LOOP ( 'NONE', ( #64790, #111241, #110936, #37589 ) ) ;
#118502=AXIS2_PLACEMENT_3D ( 'NONE', #73286, #3905, #13056 ) ;
#118503=FACE_OUTER_BOUND ( 'NONE', #53233, .T. ) ;
#118504=AXIS2_PLACEMENT_3D ( 'NONE', #74049, #123771, #45241 ) ;
#118505=ORIENTED_EDGE ( 'NONE', *, *, #110620, .F. ) ;
#118506=CARTESIAN_POINT ( 'NONE',  ( 0.8499999999999536815, 2.500000000000000000, 5.902370205355745192 ) ) ;
#118507=CARTESIAN_POINT ( 'NONE',  ( 87.50000000000002842, -6.761363245278262823, -3.308765358479924590 ) ) ;
#118508=DIRECTION ( 'NONE',  ( 0.000000000000000000, 1.000000000000000000, 0.000000000000000000 ) ) ;
#118509=VECTOR ( 'NONE', #91338, 1000.000000000000000 ) ;
#118510=CONICAL_SURFACE ( 'NONE', #103858, 0.09999999999999982514, 0.003490658503988666988 ) ;
#118511=LINE ( 'NONE', #129016, #32032 ) ;
#118512=VERTEX_POINT ( 'NONE', #81100 ) ;
#118513=LINE ( 'NONE', #108052, #112329 ) ;
#118514=DIRECTION ( 'NONE',  ( -0.000000000000000000, -1.000000000000000000, -0.000000000000000000 ) ) ;
#118516=DIRECTION ( 'NONE',  ( 0.000000000000000000, 0.000000000000000000, -1.000000000000000000 ) ) ;
#118517=DIRECTION ( 'NONE',  ( 0.000000000000000000, 1.000000000000000000, 0.000000000000000000 ) ) ;
#118519=VERTEX_POINT ( 'NONE', #51643 ) ;
#118520=EDGE_LOOP ( 'NONE', ( #103150, #30173 ) ) ;
#118521=CARTESIAN_POINT ( 'NONE',  ( 13.74999999999989519, 12.50000000000000000, -2.922977105672691422 ) ) ;
#118522=ORIENTED_EDGE ( 'NONE', *, *, #109077, .T. ) ;
#118523=DIRECTION ( 'NONE',  ( -0.000000000000000000, -1.000000000000000000, -0.000000000000000000 ) ) ;
#118524=ORIENTED_EDGE ( 'NONE', *, *, #92999, .T. ) ;
#118525=ORIENTED_EDGE ( 'NONE', *, *, #7248, .T. ) ;
#118526=VERTEX_POINT ( 'NONE', #102020 ) ;
#118527=AXIS2_PLACEMENT_3D ( 'NONE', #46898, #48180, #107083 ) ;
#118528=LINE ( 'NONE', #38722, #93882 ) ;
#118529=DIRECTION ( 'NONE',  ( 0.000000000000000000, 0.000000000000000000, 1.000000000000000000 ) ) ;
#118530=EDGE_CURVE ( 'NONE', #119523, #28738, #2501, .T. ) ;
#118531=CARTESIAN_POINT ( 'NONE',  ( 10.19999999999991225, 2.500000000000000000, 3.883716857408420431 ) ) ;
#118532=CARTESIAN_POINT ( 'NONE',  ( -8.750000000000005329, 12.50000000000000000, 5.802370205355744659 ) ) ;
#118534=DIRECTION ( 'NONE',  ( -4.274815082592931898E-19, -0.9999939076577903929, -0.003490651415223739937 ) ) ;
#118535=FACE_OUTER_BOUND ( 'NONE', #94392, .T. ) ;
#118536=EDGE_CURVE ( 'NONE', #77736, #41455, #101735, .T. ) ;
#118537=EDGE_CURVE ( 'NONE', #52488, #88829, #99692, .T. ) ;
#118538=LINE ( 'NONE', #7289, #49796 ) ;
#118539=EDGE_LOOP ( 'NONE', ( #58542, #128824 ) ) ;
#118540=AXIS2_PLACEMENT_3D ( 'NONE', #57528, #56846, #17578 ) ;
#118541=ORIENTED_EDGE ( 'NONE', *, *, #30251, .T. ) ;
#118542=ORIENTED_EDGE ( 'NONE', *, *, #95975, .F. ) ;
#118543=CIRCLE ( 'NONE', #20258, 0.1000000000000000472 ) ;
#118544=EDGE_CURVE ( 'NONE', #91624, #103089, #109913, .T. ) ;
#118546=EDGE_CURVE ( 'NONE', #66767, #83529, #71928, .T. ) ;
#118547=ORIENTED_EDGE ( 'NONE', *, *, #48211, .T. ) ;
#118548=VERTEX_POINT ( 'NONE', #49715 ) ;
#118549=EDGE_CURVE ( 'NONE', #8339, #58961, #1467, .T. ) ;
#118550=DIRECTION ( 'NONE',  ( -0.000000000000000000, 1.000000000000000000, -0.000000000000000000 ) ) ;
#118551=AXIS2_PLACEMENT_3D ( 'NONE', #8477, #66756, #48418 ) ;
#118552=CIRCLE ( 'NONE', #126883, 0.06509327318403745899 ) ;
#118553=DIRECTION ( 'NONE',  ( 0.000000000000000000, 0.000000000000000000, -1.000000000000000000 ) ) ;
#118554=DIRECTION ( 'NONE',  ( -4.274815082592931898E-19, -0.9999939076577903929, -0.003490651415223739937 ) ) ;
#118555=FACE_OUTER_BOUND ( 'NONE', #115209, .T. ) ;
#118556=FACE_OUTER_BOUND ( 'NONE', #56303, .T. ) ;
#118557=ORIENTED_EDGE ( 'NONE', *, *, #84010, .T. ) ;
#118558=CARTESIAN_POINT ( 'NONE',  ( 13.34999999999990017, 2.500000000000000000, 2.957883832488649389 ) ) ;
#118559=CIRCLE ( 'NONE', #68382, 0.06509327318403745899 ) ;
#118560=EDGE_LOOP ( 'NONE', ( #10325, #77222, #937, #1607 ) ) ;
#118561=CARTESIAN_POINT ( 'NONE',  ( 1.699999999999951994, 12.50000000000000000, -0.06509327318403970719 ) ) ;
#118562=CIRCLE ( 'NONE', #74756, 0.1000000000000002554 ) ;
#118563=EDGE_LOOP ( 'NONE', ( #86661, #61314, #68788, #75227 ) ) ;
#118564=DIRECTION ( 'NONE',  ( -0.000000000000000000, -1.000000000000000000, -0.000000000000000000 ) ) ;
#118565=VERTEX_POINT ( 'NONE', #20238 ) ;
#118566=VERTEX_POINT ( 'NONE', #50340 ) ;
#118567=LINE ( 'NONE', #68828, #119261 ) ;
#118568=CARTESIAN_POINT ( 'NONE',  ( -14.19999999999998685, 2.500000000000000000, -0.1000000000000001166 ) ) ;
#118569=CARTESIAN_POINT ( 'NONE',  ( 13.34999999999989662, 2.500000000000000000, -1.372243186433550033 ) ) ;
#118570=DIRECTION ( 'NONE',  ( 0.000000000000000000, 0.000000000000000000, 1.000000000000000000 ) ) ;
#118571=CARTESIAN_POINT ( 'NONE',  ( 3.349999999999941025, 12.50000000000000000, 7.188010851410848723 ) ) ;
#118572=EDGE_LOOP ( 'NONE', ( #39510, #42676 ) ) ;
#118573=LINE ( 'NONE', #68837, #18595 ) ;
#118574=CARTESIAN_POINT ( 'NONE',  ( -3.300000000000028244, 2.500000000000000000, 4.330127018922196314 ) ) ;
#118575=DIRECTION ( 'NONE',  ( 0.000000000000000000, 0.000000000000000000, 1.000000000000000000 ) ) ;
#118576=CARTESIAN_POINT ( 'NONE',  ( -9.600000000000006750, 2.500000000000000000, 5.022947341949748790 ) ) ;
#118577=CIRCLE ( 'NONE', #3570, 0.09999999999999982514 ) ;
#118578=CONICAL_SURFACE ( 'NONE', #24590, 0.09999999999999982514, 0.003490658503988666988 ) ;
#118579=DIRECTION ( 'NONE',  ( 0.000000000000000000, 1.000000000000000000, 0.000000000000000000 ) ) ;
#118580=ORIENTED_EDGE ( 'NONE', *, *, #42569, .T. ) ;
#118581=AXIS2_PLACEMENT_3D ( 'NONE', #5568, #59880, #98460 ) ;
#118582=ORIENTED_EDGE ( 'NONE', *, *, #110052, .T. ) ;
#118583=EDGE_CURVE ( 'NONE', #96946, #41415, #110542, .T. ) ;
#118584=DIRECTION ( 'NONE',  ( -0.000000000000000000, -1.000000000000000000, -0.000000000000000000 ) ) ;
#118585=EDGE_CURVE ( 'NONE', #79172, #2432, #90241, .T. ) ;
#118586=AXIS2_PLACEMENT_3D ( 'NONE', #90654, #989, #121402 ) ;
#118587=EDGE_CURVE ( 'NONE', #13065, #92822, #78863, .T. ) ;
#118588=ORIENTED_EDGE ( 'NONE', *, *, #73862, .T. ) ;
#118589=CIRCLE ( 'NONE', #57967, 0.06509327318403745899 ) ;
#118590=LINE ( 'NONE', #19763, #48749 ) ;
#118591=CARTESIAN_POINT ( 'NONE',  ( 4.999999999999936939, 2.500000000000000000, -3.737306695894649700 ) ) ;
#118592=AXIS2_PLACEMENT_3D ( 'NONE', #95868, #37603, #36323 ) ;
#118593=AXIS2_PLACEMENT_3D ( 'NONE', #596, #60826, #110560 ) ;
#118594=EDGE_CURVE ( 'NONE', #91624, #74274, #120610, .T. ) ;
#118595=ORIENTED_EDGE ( 'NONE', *, *, #72742, .T. ) ;
#118597=DIRECTION ( 'NONE',  ( 0.000000000000000000, 1.000000000000000000, 0.000000000000000000 ) ) ;
#118598=CIRCLE ( 'NONE', #70483, 0.1000000000000000472 ) ;
#118599=EDGE_CURVE ( 'NONE', #113021, #93976, #51000, .T. ) ;
#118600=DIRECTION ( 'NONE',  ( 0.000000000000000000, 0.000000000000000000, 1.000000000000000000 ) ) ;
#118601=DIRECTION ( 'NONE',  ( 0.000000000000000000, 1.000000000000000000, 0.000000000000000000 ) ) ;
#118602=ORIENTED_EDGE ( 'NONE', *, *, #3917, .F. ) ;
#118603=ADVANCED_FACE ( 'NONE', ( #22188 ), #121010, .T. ) ;
#118604=EDGE_CURVE ( 'NONE', #84227, #87575, #32894, .T. ) ;
#118605=AXIS2_PLACEMENT_3D ( 'NONE', #72992, #112914, #23234 ) ;
#118606=AXIS2_PLACEMENT_3D ( 'NONE', #114328, #2420, #52190 ) ;
#118607=ADVANCED_FACE ( 'NONE', ( #114405 ), #122657, .T. ) ;
#118608=DIRECTION ( 'NONE',  ( 0.000000000000000000, 0.000000000000000000, -1.000000000000000000 ) ) ;
#118609=EDGE_LOOP ( 'NONE', ( #124673, #66918 ) ) ;
#118611=DIRECTION ( 'NONE',  ( -0.000000000000000000, 1.000000000000000000, -0.000000000000000000 ) ) ;
#118612=DIRECTION ( 'NONE',  ( 0.000000000000000000, -0.9999939076577903929, 0.003490651415223739937 ) ) ;
#118613=EDGE_CURVE ( 'NONE', #6029, #41590, #13622, .T. ) ;
#118614=CARTESIAN_POINT ( 'NONE',  ( 11.89999999999990798, 2.500000000000000000, -4.676537180435977881 ) ) ;
#118615=ORIENTED_EDGE ( 'NONE', *, *, #70981, .T. ) ;
#118616=DIRECTION ( 'NONE',  ( 0.000000000000000000, 0.000000000000000000, 1.000000000000000000 ) ) ;
#118617=VERTEX_POINT ( 'NONE', #113116 ) ;
#118618=CARTESIAN_POINT ( 'NONE',  ( -2.700000000000030376, 12.50000000000000000, 3.918623584224383727 ) ) ;
#118619=CARTESIAN_POINT ( 'NONE',  ( -8.100000000000010303, 2.500000000000000000, 4.083716857408421497 ) ) ;
#118620=AXIS2_PLACEMENT_3D ( 'NONE', #115764, #66022, #56192 ) ;
#118621=CARTESIAN_POINT ( 'NONE',  ( 1.449999999999951772, 2.500000000000000000, -6.048780366869526581 ) ) ;
#118622=VERTEX_POINT ( 'NONE', #17304 ) ;
#118623=CARTESIAN_POINT ( 'NONE',  ( 8.749999999999957367, 2.500000000000000000, -6.395190528383301931 ) ) ;
#118625=ORIENTED_EDGE ( 'NONE', *, *, #81203, .T. ) ;
#118626=CARTESIAN_POINT ( 'NONE',  ( -10.20000000000000462, 2.500000000000000000, 0.3464101615137735735 ) ) ;
#118627=ORIENTED_EDGE ( 'NONE', *, *, #82565, .T. ) ;
#118628=DIRECTION ( 'NONE',  ( 0.000000000000000000, 1.000000000000000000, 0.000000000000000000 ) ) ;
#118629=AXIS2_PLACEMENT_3D ( 'NONE', #68956, #89243, #57205 ) ;
#118630=VECTOR ( 'NONE', #35551, 1000.000000000000000 ) ;
#118631=ORIENTED_EDGE ( 'NONE', *, *, #67383, .F. ) ;
#118632=CARTESIAN_POINT ( 'NONE',  ( 2.299999999999948752, 12.50000000000000000, 0.3464101615137735735 ) ) ;
#118633=DIRECTION ( 'NONE',  ( 0.000000000000000000, 0.000000000000000000, 1.000000000000000000 ) ) ;
#118634=ORIENTED_EDGE ( 'NONE', *, *, #76940, .T. ) ;
#118635=ORIENTED_EDGE ( 'NONE', *, *, #84580, .F. ) ;
#118636=DIRECTION ( 'NONE',  ( 0.000000000000000000, 0.000000000000000000, -1.000000000000000000 ) ) ;
#118637=CARTESIAN_POINT ( 'NONE',  ( 11.64999999999990798, 12.50000000000000000, 7.188010851410848723 ) ) ;
#118638=VERTEX_POINT ( 'NONE', #127304 ) ;
#118640=DIRECTION ( 'NONE',  ( 0.000000000000000000, 0.000000000000000000, -1.000000000000000000 ) ) ;
#118641=AXIS2_PLACEMENT_3D ( 'NONE', #20511, #90521, #40811 ) ;
#118642=EDGE_CURVE ( 'NONE', #90643, #18500, #11935, .T. ) ;
#118643=AXIS2_PLACEMENT_3D ( 'NONE', #102278, #42067, #121913 ) ;
#118644=DIRECTION ( 'NONE',  ( -0.000000000000000000, -1.000000000000000000, -0.000000000000000000 ) ) ;
#118645=DIRECTION ( 'NONE',  ( 0.000000000000000000, 1.000000000000000000, 0.000000000000000000 ) ) ;
#118646=DIRECTION ( 'NONE',  ( 0.000000000000000000, 0.000000000000000000, 1.000000000000000000 ) ) ;
#118647=DIRECTION ( 'NONE',  ( -0.000000000000000000, 1.000000000000000000, -0.000000000000000000 ) ) ;
#118648=CARTESIAN_POINT ( 'NONE',  ( 3.299999999999942979, 2.500000000000000000, 4.330127018922196314 ) ) ;
#118649=VERTEX_POINT ( 'NONE', #102650 ) ;
#118650=ORIENTED_EDGE ( 'NONE', *, *, #21456, .F. ) ;
#118651=ORIENTED_EDGE ( 'NONE', *, *, #12295, .F. ) ;
#118652=ORIENTED_EDGE ( 'NONE', *, *, #46817, .F. ) ;
#118653=DIRECTION ( 'NONE',  ( -0.000000000000000000, 1.000000000000000000, -0.000000000000000000 ) ) ;
#118654=CARTESIAN_POINT ( 'NONE',  ( 2.299999999999946976, 12.50000000000000000, 4.741630453620009789 ) ) ;
#118655=AXIS2_PLACEMENT_3D ( 'NONE', #72236, #90562, #121968 ) ;
#118656=DIRECTION ( 'NONE',  ( -0.000000000000000000, -1.000000000000000000, -0.000000000000000000 ) ) ;
#118657=VERTEX_POINT ( 'NONE', #3813 ) ;
#118658=EDGE_CURVE ( 'NONE', #89337, #40173, #57269, .T. ) ;
#118659=FACE_BOUND ( 'NONE', #51213, .T. ) ;
#118660=ORIENTED_EDGE ( 'NONE', *, *, #20089, .F. ) ;
#118661=DIRECTION ( 'NONE',  ( 0.000000000000000000, -0.9999939076577903929, 0.003490651415223739937 ) ) ;
#118662=CARTESIAN_POINT ( 'NONE',  ( -15.19999999999998153, 2.500000000000000000, -0.4464101615137759382 ) ) ;
#118663=DIRECTION ( 'NONE',  ( 0.000000000000000000, -0.000000000000000000, 1.000000000000000000 ) ) ;
#118664=AXIS2_PLACEMENT_3D ( 'NONE', #129119, #60376, #100278 ) ;
#118666=CARTESIAN_POINT ( 'NONE',  ( -13.94999999999998863, 12.50000000000000000, -1.883746621131361376 ) ) ;
#118667=CARTESIAN_POINT ( 'NONE',  ( 3.749999999999944045, 12.50000000000000000, -7.122917578226816815 ) ) ;
#118668=ORIENTED_EDGE ( 'NONE', *, *, #90177, .T. ) ;
#118669=FACE_OUTER_BOUND ( 'NONE', #125539, .T. ) ;
#118670=CARTESIAN_POINT ( 'NONE',  ( -6.700000000000019718, 2.500000000000000000, -4.230127018922201998 ) ) ;
#118672=CIRCLE ( 'NONE', #81037, 0.09999999999999982514 ) ;
#118673=CARTESIAN_POINT ( 'NONE',  ( 10.84999999999991260, 2.500000000000000000, -2.857883832488653741 ) ) ;
#118674=ORIENTED_EDGE ( 'NONE', *, *, #92723, .T. ) ;
#118676=ORIENTED_EDGE ( 'NONE', *, *, #52356, .T. ) ;
#118678=ORIENTED_EDGE ( 'NONE', *, *, #11133, .F. ) ;
#118679=CARTESIAN_POINT ( 'NONE',  ( 12.69999999999990159, 12.50000000000000000, -3.983716857408426293 ) ) ;
#118680=DIRECTION ( 'NONE',  ( -1.000000000000000000, 0.000000000000000000, 0.000000000000000000 ) ) ;
#118681=ORIENTED_EDGE ( 'NONE', *, *, #23538, .F. ) ;
#118682=ORIENTED_EDGE ( 'NONE', *, *, #8213, .T. ) ;
#118683=AXIS2_PLACEMENT_3D ( 'NONE', #95173, #5480, #115421 ) ;
#118684=VERTEX_POINT ( 'NONE', #27156 ) ;
#118685=DIRECTION ( 'NONE',  ( 0.000000000000000000, 0.000000000000000000, -1.000000000000000000 ) ) ;
#118686=AXIS2_PLACEMENT_3D ( 'NONE', #38353, #39017, #77602 ) ;
#118687=CIRCLE ( 'NONE', #5798, 0.09999999999999982514 ) ;
#118688=ADVANCED_FACE ( 'NONE', ( #53565 ), #85093, .T. ) ;
#118689=DIRECTION ( 'NONE',  ( -4.274815082592931898E-19, -0.9999939076577903929, -0.003490651415223739937 ) ) ;
#118690=CARTESIAN_POINT ( 'NONE',  ( 2.099999999999949463, 12.50000000000000000, -3.637306695894650055 ) ) ;
#118691=DIRECTION ( 'NONE',  ( 0.000000000000000000, 0.000000000000000000, -1.000000000000000000 ) ) ;
#118692=DIRECTION ( 'NONE',  ( 0.000000000000000000, 0.000000000000000000, 1.000000000000000000 ) ) ;
#118693=CARTESIAN_POINT ( 'NONE',  ( 8.099999999999921485, 2.500000000000000000, 0.3464101615137735735 ) ) ;
#118694=CARTESIAN_POINT ( 'NONE',  ( -6.650000000000019007, 2.500000000000000000, -1.472243186433550122 ) ) ;
#118695=CIRCLE ( 'NONE', #95721, 0.09999999999999982514 ) ;
#118696=VERTEX_POINT ( 'NONE', #4423 ) ;
#118697=EDGE_CURVE ( 'NONE', #101221, #60915, #64163, .T. ) ;
#118698=DIRECTION ( 'NONE',  ( 0.000000000000000000, 0.000000000000000000, 1.000000000000000000 ) ) ;
#118699=EDGE_LOOP ( 'NONE', ( #7868, #38611 ) ) ;
#118700=AXIS2_PLACEMENT_3D ( 'NONE', #90010, #110316, #59301 ) ;
#118701=ORIENTED_EDGE ( 'NONE', *, *, #62355, .F. ) ;
#118702=VERTEX_POINT ( 'NONE', #92854 ) ;
#118703=EDGE_CURVE ( 'NONE', #50242, #13848, #26520, .T. ) ;
#118704=FACE_OUTER_BOUND ( 'NONE', #28881, .T. ) ;
#118705=ADVANCED_FACE ( 'NONE', ( #43125 ), #7508, .T. ) ;
#118706=EDGE_CURVE ( 'NONE', #62255, #10677, #95570, .T. ) ;
#118707=ORIENTED_EDGE ( 'NONE', *, *, #79246, .T. ) ;
#118708=EDGE_CURVE ( 'NONE', #41901, #70057, #32800, .T. ) ;
#118709=EDGE_CURVE ( 'NONE', #55123, #85856, #45400, .T. ) ;
#118711=CARTESIAN_POINT ( 'NONE',  ( -2.100000000000034284, 2.500000000000000000, -0.1000000000000023925 ) ) ;
#118712=DIRECTION ( 'NONE',  ( 0.000000000000000000, -0.000000000000000000, 1.000000000000000000 ) ) ;
#118713=DIRECTION ( 'NONE',  ( 0.000000000000000000, 0.000000000000000000, 1.000000000000000000 ) ) ;
#118714=CARTESIAN_POINT ( 'NONE',  ( -8.749999999999976907, 2.500000000000000000, -6.495190528383297135 ) ) ;
#118715=CARTESIAN_POINT ( 'NONE',  ( -1.650000000000034772, 2.500000000000000000, 1.472243186433545459 ) ) ;
#118716=EDGE_CURVE ( 'NONE', #47149, #120218, #129045, .T. ) ;
#118717=VERTEX_POINT ( 'NONE', #16665 ) ;
#118718=CARTESIAN_POINT ( 'NONE',  ( -4.800000000000024691, 2.500000000000000000, 4.776537180435972196 ) ) ;
#118719=ADVANCED_FACE ( 'NONE', ( #123573 ), #34587, .T. ) ;
#118720=ADVANCED_FACE ( 'NONE', ( #73843 ), #105937, .T. ) ;
#118721=ORIENTED_EDGE ( 'NONE', *, *, #49464, .F. ) ;
#118722=DIRECTION ( 'NONE',  ( 0.000000000000000000, 0.000000000000000000, 1.000000000000000000 ) ) ;
#118723=ORIENTED_EDGE ( 'NONE', *, *, #30089, .T. ) ;
#118724=CARTESIAN_POINT ( 'NONE',  ( 1.049999999999953637, 2.500000000000000000, -1.718653347947326049 ) ) ;
#118725=DIRECTION ( 'NONE',  ( 0.000000000000000000, 1.000000000000000000, 0.000000000000000000 ) ) ;
#118726=EDGE_LOOP ( 'NONE', ( #70816, #101398, #67072, #72244 ) ) ;
#118727=DIRECTION ( 'NONE',  ( 0.000000000000000000, 0.000000000000000000, -1.000000000000000000 ) ) ;
#118728=AXIS2_PLACEMENT_3D ( 'NONE', #73742, #24023, #14804 ) ;
#118729=LINE ( 'NONE', #59185, #74996 ) ;
#118730=ORIENTED_EDGE ( 'NONE', *, *, #87616, .F. ) ;
#118731=VECTOR ( 'NONE', #5998, 1000.000000000000000 ) ;
#118732=AXIS2_PLACEMENT_3D ( 'NONE', #96369, #6683, #9942 ) ;
#118733=CARTESIAN_POINT ( 'NONE',  ( -9.150000000000005684, 12.50000000000000000, 6.430097255199259010 ) ) ;
#118734=ORIENTED_EDGE ( 'NONE', *, *, #30650, .T. ) ;
#118735=EDGE_LOOP ( 'NONE', ( #89199, #128845, #98678, #79237 ) ) ;
#118736=CARTESIAN_POINT ( 'NONE',  ( 6.899999999999928413, 2.500000000000000000, -3.983716857408426293 ) ) ;
#118737=PLANE ( 'NONE',  #43015 ) ;
#118738=CARTESIAN_POINT ( 'NONE',  ( -6.250000000000019540, 2.500000000000000000, -7.288010851410854585 ) ) ;
#118739=CARTESIAN_POINT ( 'NONE',  ( -12.94999999999999218, 12.50000000000000000, 2.165063509461101265 ) ) ;
#118740=CIRCLE ( 'NONE', #60178, 0.1000000000000002554 ) ;
#118741=PLANE ( 'NONE',  #52029 ) ;
#118742=AXIS2_PLACEMENT_3D ( 'NONE', #23593, #121785, #43900 ) ;
#118743=ORIENTED_EDGE ( 'NONE', *, *, #63912, .T. ) ;
#118744=DIRECTION ( 'NONE',  ( 0.000000000000000000, 0.000000000000000000, 1.000000000000000000 ) ) ;
#118745=EDGE_CURVE ( 'NONE', #17419, #27445, #103884, .T. ) ;
#118746=ORIENTED_EDGE ( 'NONE', *, *, #25025, .F. ) ;
#118747=CARTESIAN_POINT ( 'NONE',  ( 5.649999999999934630, 2.500000000000000000, -2.411473670974877859 ) ) ;
#118748=DIRECTION ( 'NONE',  ( 0.000000000000000000, 0.000000000000000000, -1.000000000000000000 ) ) ;
#118749=CIRCLE ( 'NONE', #122963, 0.06509327318403745899 ) ;
#118750=ADVANCED_FACE ( 'NONE', ( #116816 ), #30748, .T. ) ;
#118751=EDGE_LOOP ( 'NONE', ( #42095, #13408, #100209, #15172 ) ) ;
#118752=DIRECTION ( 'NONE',  ( 0.000000000000000000, 0.000000000000000000, -1.000000000000000000 ) ) ;
#118753=DIRECTION ( 'NONE',  ( 0.000000000000000000, 0.000000000000000000, -1.000000000000000000 ) ) ;
#118754=CARTESIAN_POINT ( 'NONE',  ( -6.650000000000018119, 12.50000000000000000, -6.495190528383302464 ) ) ;
#118756=CARTESIAN_POINT ( 'NONE',  ( -8.750000000000010658, 2.500000000000000000, -1.472243186433550122 ) ) ;
#118757=CARTESIAN_POINT ( 'NONE',  ( -5.650000000000019895, 2.500000000000000000, 1.818653347947321475 ) ) ;
#118758=VERTEX_POINT ( 'NONE', #40876 ) ;
#118759=ADVANCED_FACE ( 'NONE', ( #29114 ), #108291, .T. ) ;
#118760=VECTOR ( 'NONE', #81075, 1000.000000000000000 ) ;
#118761=CARTESIAN_POINT ( 'NONE',  ( 0.1999999999999627909, 2.500000000000000000, 0.3464101615137758494 ) ) ;
#118762=EDGE_CURVE ( 'NONE', #28400, #43992, #66221, .T. ) ;
#118763=CARTESIAN_POINT ( 'NONE',  ( -1.250000000000001554, 12.50000000000000000, 2.230156782645134950 ) ) ;
#118764=DIRECTION ( 'NONE',  ( -0.000000000000000000, -1.000000000000000000, -0.000000000000000000 ) ) ;
#118765=AXIS2_PLACEMENT_3D ( 'NONE', #121275, #23729, #32922 ) ;
#118766=VECTOR ( 'NONE', #49985, 1000.000000000000000 ) ;
#118767=ORIENTED_EDGE ( 'NONE', *, *, #3386, .T. ) ;
#118768=CIRCLE ( 'NONE', #76911, 0.06509327318403745899 ) ;
#118769=EDGE_CURVE ( 'NONE', #79642, #8138, #118543, .T. ) ;
#118770=DIRECTION ( 'NONE',  ( -0.000000000000000000, 1.000000000000000000, -0.000000000000000000 ) ) ;
#118771=AXIS2_PLACEMENT_3D ( 'NONE', #51174, #21707, #10570 ) ;
#118772=ORIENTED_EDGE ( 'NONE', *, *, #102587, .T. ) ;
#118773=EDGE_LOOP ( 'NONE', ( #21924, #21033 ) ) ;
#118774=DIRECTION ( 'NONE',  ( 0.000000000000000000, 0.000000000000000000, 1.000000000000000000 ) ) ;
#118775=VECTOR ( 'NONE', #24351, 1000.000000000000000 ) ;
#118776=EDGE_LOOP ( 'NONE', ( #126802, #121887, #3966, #71922 ) ) ;
#118777=PLANE ( 'NONE',  #100926 ) ;
#118778=CARTESIAN_POINT ( 'NONE',  ( -2.900000000000029221, 2.500000000000000000, -2.276824562219559311E-15 ) ) ;
#118779=VERTEX_POINT ( 'NONE', #58567 ) ;
#118780=DIRECTION ( 'NONE',  ( 0.000000000000000000, 0.000000000000000000, 1.000000000000000000 ) ) ;
#118781=DIRECTION ( 'NONE',  ( 0.000000000000000000, 0.000000000000000000, -1.000000000000000000 ) ) ;
#118782=EDGE_LOOP ( 'NONE', ( #66408, #22345 ) ) ;
#118783=DIRECTION ( 'NONE',  ( -4.274815082592931898E-19, -0.9999939076577903929, -0.003490651415223739937 ) ) ;
#118784=CONICAL_SURFACE ( 'NONE', #81146, 0.09999999999999982514, 0.003490658503988666988 ) ;
#118785=LINE ( 'NONE', #17341, #101146 ) ;
#118786=EDGE_CURVE ( 'NONE', #46382, #38829, #89937, .T. ) ;
#118787=ORIENTED_EDGE ( 'NONE', *, *, #95679, .T. ) ;
#118788=AXIS2_PLACEMENT_3D ( 'NONE', #34219, #14542, #54477 ) ;
#118789=CIRCLE ( 'NONE', #91606, 0.1000000000000002554 ) ;
#118790=ORIENTED_EDGE ( 'NONE', *, *, #41618, .T. ) ;
#118791=ORIENTED_EDGE ( 'NONE', *, *, #100856, .F. ) ;
#118792=DIRECTION ( 'NONE',  ( -0.000000000000000000, 1.000000000000000000, -0.000000000000000000 ) ) ;
#118793=DIRECTION ( 'NONE',  ( 0.000000000000000000, 1.000000000000000000, 0.000000000000000000 ) ) ;
#118794=DIRECTION ( 'NONE',  ( -0.000000000000000000, 1.000000000000000000, -0.000000000000000000 ) ) ;
#118795=FACE_BOUND ( 'NONE', #63992, .T. ) ;
#118796=ORIENTED_EDGE ( 'NONE', *, *, #71257, .T. ) ;
#118798=DIRECTION ( 'NONE',  ( 0.000000000000000000, 0.000000000000000000, -1.000000000000000000 ) ) ;
#118799=ORIENTED_EDGE ( 'NONE', *, *, #64602, .T. ) ;
#118800=CARTESIAN_POINT ( 'NONE',  ( 1.249999999999988454, 2.500000000000000000, -2.065063509461102065 ) ) ;
#118801=CARTESIAN_POINT ( 'NONE',  ( -11.25000000000000000, 2.500000000000000000, 2.757883832488649656 ) ) ;
#118802=EDGE_CURVE ( 'NONE', #72180, #97645, #39159, .T. ) ;
#118803=DIRECTION ( 'NONE',  ( 0.000000000000000000, 1.000000000000000000, 0.000000000000000000 ) ) ;
#118804=DIRECTION ( 'NONE',  ( 0.000000000000000000, 0.000000000000000000, -1.000000000000000000 ) ) ;
#118805=CIRCLE ( 'NONE', #62392, 0.1000000000000002554 ) ;
#118806=FACE_OUTER_BOUND ( 'NONE', #81067, .T. ) ;
#118807=DIRECTION ( 'NONE',  ( 0.000000000000000000, -0.000000000000000000, 1.000000000000000000 ) ) ;
#118808=DIRECTION ( 'NONE',  ( 0.000000000000000000, 0.000000000000000000, -1.000000000000000000 ) ) ;
#118809=AXIS2_PLACEMENT_3D ( 'NONE', #24256, #61618, #91062 ) ;
#118810=VECTOR ( 'NONE', #27764, 1000.000000000000000 ) ;
#118811=VERTEX_POINT ( 'NONE', #120055 ) ;
#118812=EDGE_LOOP ( 'NONE', ( #114911, #45729 ) ) ;
#118813=VERTEX_POINT ( 'NONE', #68363 ) ;
#118814=CONICAL_SURFACE ( 'NONE', #114598, 0.1000000000000002554, 0.003490658503988666988 ) ;
#118815=AXIS2_PLACEMENT_3D ( 'NONE', #22924, #47081, #45145 ) ;
#118816=ORIENTED_EDGE ( 'NONE', *, *, #15756, .F. ) ;
#118817=VERTEX_POINT ( 'NONE', #99130 ) ;
#118818=FACE_OUTER_BOUND ( 'NONE', #74033, .T. ) ;
#118819=DIRECTION ( 'NONE',  ( -0.000000000000000000, -1.000000000000000000, -0.000000000000000000 ) ) ;
#118820=ORIENTED_EDGE ( 'NONE', *, *, #94927, .T. ) ;
#118821=ADVANCED_FACE ( 'NONE', ( #80787 ), #110145, .T. ) ;
#118822=FACE_BOUND ( 'NONE', #65979, .T. ) ;
#118823=DIRECTION ( 'NONE',  ( -4.274815082592931898E-19, -0.9999939076577903929, -0.003490651415223739937 ) ) ;
#118824=AXIS2_PLACEMENT_3D ( 'NONE', #66201, #77957, #117213 ) ;
#118825=AXIS2_PLACEMENT_3D ( 'NONE', #97616, #117890, #87782 ) ;
#118826=DIRECTION ( 'NONE',  ( 0.000000000000000000, 0.000000000000000000, -1.000000000000000000 ) ) ;
#118827=CARTESIAN_POINT ( 'NONE',  ( -7.950000000000016165, 2.500000000000000000, -6.395190528383296602 ) ) ;
#118828=CARTESIAN_POINT ( 'NONE',  ( 3.949999999999940670, 2.500000000000000000, 1.918653347947321564 ) ) ;
#118829=DIRECTION ( 'NONE',  ( 0.000000000000000000, 0.000000000000000000, 1.000000000000000000 ) ) ;
#118830=EDGE_LOOP ( 'NONE', ( #85198, #3911 ) ) ;
#118831=AXIS2_PLACEMENT_3D ( 'NONE', #94802, #88845, #59415 ) ;
#118832=VERTEX_POINT ( 'NONE', #98457 ) ;
#118833=ORIENTED_EDGE ( 'NONE', *, *, #2286, .F. ) ;
#118834=EDGE_LOOP ( 'NONE', ( #84090, #13513 ) ) ;
#118835=DIRECTION ( 'NONE',  ( -0.000000000000000000, 1.000000000000000000, -0.000000000000000000 ) ) ;
#118837=CARTESIAN_POINT ( 'NONE',  ( 4.149999999999939959, 2.500000000000000000, 2.857883832488649301 ) ) ;
#118838=ORIENTED_EDGE ( 'NONE', *, *, #17308, .F. ) ;
#118839=DIRECTION ( 'NONE',  ( 0.000000000000000000, 0.000000000000000000, 1.000000000000000000 ) ) ;
#118840=AXIS2_PLACEMENT_3D ( 'NONE', #85665, #125579, #87591 ) ;
#118841=DIRECTION ( 'NONE',  ( -0.000000000000000000, 1.000000000000000000, -0.000000000000000000 ) ) ;
#118842=ADVANCED_FACE ( 'NONE', ( #69657 ), #19928, .T. ) ;
#118843=CARTESIAN_POINT ( 'NONE',  ( 2.049999999999950084, 2.500000000000000000, -6.495190528383302464 ) ) ;
#118844=AXIS2_PLACEMENT_3D ( 'NONE', #107572, #48654, #88563 ) ;
#118846=CARTESIAN_POINT ( 'NONE',  ( 7.099999999999928590, 2.500000000000000000, 4.330127018922196314 ) ) ;
#118847=DIRECTION ( 'NONE',  ( -0.000000000000000000, -1.000000000000000000, -0.000000000000000000 ) ) ;
#118848=CIRCLE ( 'NONE', #54015, 0.06509327318403743123 ) ;
#118849=CARTESIAN_POINT ( 'NONE',  ( -5.650000000000019895, 2.500000000000000000, 6.048780366869520364 ) ) ;
#118851=CARTESIAN_POINT ( 'NONE',  ( -13.34999999999999076, 2.500000000000000000, 2.857883832488652853 ) ) ;
#118852=ADVANCED_FACE ( 'NONE', ( #109595 ), #8792, .T. ) ;
#118853=AXIS2_PLACEMENT_3D ( 'NONE', #117743, #97482, #126951 ) ;
#118854=VERTEX_POINT ( 'NONE', #48745 ) ;
#118855=ORIENTED_EDGE ( 'NONE', *, *, #59570, .F. ) ;
#118856=FACE_OUTER_BOUND ( 'NONE', #116742, .T. ) ;
#118858=DIRECTION ( 'NONE',  ( 0.000000000000000000, -0.9999939076577903929, 0.003490651415223739937 ) ) ;
#118859=DIRECTION ( 'NONE',  ( -0.000000000000000000, 1.000000000000000000, -0.000000000000000000 ) ) ;
#118860=EDGE_CURVE ( 'NONE', #58034, #69008, #80131, .T. ) ;
#118861=EDGE_CURVE ( 'NONE', #85654, #116200, #40210, .T. ) ;
#118862=EDGE_CURVE ( 'NONE', #22575, #75000, #16210, .T. ) ;
#118864=CONICAL_SURFACE ( 'NONE', #89525, 0.1000000000000000472, 0.003490658503988666988 ) ;
#118865=EDGE_LOOP ( 'NONE', ( #37162, #1414 ) ) ;
#118866=DIRECTION ( 'NONE',  ( 0.000000000000000000, 0.000000000000000000, -1.000000000000000000 ) ) ;
#118867=AXIS2_PLACEMENT_3D ( 'NONE', #26212, #66125, #119103 ) ;
#118868=CARTESIAN_POINT ( 'NONE',  ( 3.349999999999944578, 12.50000000000000000, -1.537336459617587581 ) ) ;
#118869=ADVANCED_FACE ( 'NONE', ( #78860 ), #60079, .T. ) ;
#118870=DIRECTION ( 'NONE',  ( 0.000000000000000000, 0.000000000000000000, -1.000000000000000000 ) ) ;
#118871=EDGE_LOOP ( 'NONE', ( #23432, #104368, #64268, #99799 ) ) ;
#118872=EDGE_CURVE ( 'NONE', #35274, #86441, #106122, .T. ) ;
#118873=CARTESIAN_POINT ( 'NONE',  ( 9.999999999999914735, 12.50000000000000000, 0.7579135962115869374 ) ) ;
#118874=AXIS2_PLACEMENT_3D ( 'NONE', #44622, #102881, #34825 ) ;
#118875=EDGE_CURVE ( 'NONE', #27907, #44544, #41298, .T. ) ;
#118876=VERTEX_POINT ( 'NONE', #110858 ) ;
#118877=DIRECTION ( 'NONE',  ( -4.274815082592931898E-19, -0.9999939076577903929, -0.003490651415223739937 ) ) ;
#118878=EDGE_CURVE ( 'NONE', #109309, #118684, #91237, .T. ) ;
#118879=EDGE_CURVE ( 'NONE', #42202, #4198, #93512, .T. ) ;
#118880=VERTEX_POINT ( 'NONE', #13302 ) ;
#118881=CARTESIAN_POINT ( 'NONE',  ( -11.25000000000000178, 2.500000000000000000, -5.802370205355746435 ) ) ;
#118882=CONICAL_SURFACE ( 'NONE', #108693, 0.1000000000000002554, 0.003490658503988666988 ) ;
#118883=CARTESIAN_POINT ( 'NONE',  ( 12.04999999999990479, 2.500000000000000000, -6.595190528383302109 ) ) ;
#118884=CARTESIAN_POINT ( 'NONE',  ( 4.149999999999941735, 2.500000000000000000, -2.957883832488653830 ) ) ;
#118885=AXIS2_PLACEMENT_3D ( 'NONE', #57981, #57329, #118175 ) ;
#118886=DIRECTION ( 'NONE',  ( -0.000000000000000000, -1.000000000000000000, -0.000000000000000000 ) ) ;
#118887=EDGE_CURVE ( 'NONE', #80402, #122002, #101923, .T. ) ;
#118888=EDGE_LOOP ( 'NONE', ( #66503, #34187, #8392, #77004 ) ) ;
#118889=CARTESIAN_POINT ( 'NONE',  ( -11.64999999999999858, 12.50000000000000000, -1.407149913249508666 ) ) ;
#118890=VECTOR ( 'NONE', #3555, 1000.000000000000000 ) ;
#118891=EDGE_LOOP ( 'NONE', ( #17987, #126019, #51565, #99051 ) ) ;
#118892=ORIENTED_EDGE ( 'NONE', *, *, #121225, .F. ) ;
#118893=CARTESIAN_POINT ( 'NONE',  ( -4.150000000000028777, 12.50000000000000000, -5.802370205355749988 ) ) ;
#118894=PLANE ( 'NONE',  #17746 ) ;
#118895=DIRECTION ( 'NONE',  ( 0.000000000000000000, 0.000000000000000000, 1.000000000000000000 ) ) ;
#118896=DIRECTION ( 'NONE',  ( -0.000000000000000000, 1.000000000000000000, -0.000000000000000000 ) ) ;
#118897=DIRECTION ( 'NONE',  ( 0.000000000000000000, 1.000000000000000000, 0.000000000000000000 ) ) ;
#118898=FACE_OUTER_BOUND ( 'NONE', #73610, .T. ) ;
#118899=DIRECTION ( 'NONE',  ( 0.000000000000000000, 1.000000000000000000, 0.000000000000000000 ) ) ;
#118900=CARTESIAN_POINT ( 'NONE',  ( 8.749999999999923617, 12.50000000000000000, -7.188010851410854052 ) ) ;
#118901=FACE_OUTER_BOUND ( 'NONE', #84851, .T. ) ;
#118902=CIRCLE ( 'NONE', #77134, 0.06509327318403745899 ) ;
#118903=CONICAL_SURFACE ( 'NONE', #24910, 0.09999999999999982514, 0.003490658503988666988 ) ;
#118904=VECTOR ( 'NONE', #89911, 1000.000000000000000 ) ;
#118905=EDGE_LOOP ( 'NONE', ( #99091, #125746, #83656, #60588 ) ) ;
#118906=CIRCLE ( 'NONE', #54064, 0.06509327318403745899 ) ;
#118907=CARTESIAN_POINT ( 'NONE',  ( 2.299999999999947864, 12.50000000000000000, 3.983716857408420964 ) ) ;
#118908=CARTESIAN_POINT ( 'NONE',  ( 1.449999999999951328, 2.500000000000000000, -1.718653347947326049 ) ) ;
#118909=DIRECTION ( 'NONE',  ( -4.274815082592931898E-19, -0.9999939076577903929, -0.003490651415223739937 ) ) ;
#118910=FACE_OUTER_BOUND ( 'NONE', #81428, .T. ) ;
#118911=CARTESIAN_POINT ( 'NONE',  ( -1.650000000000034328, 2.500000000000000000, -2.757883832488654097 ) ) ;
#118912=CIRCLE ( 'NONE', #6031, 0.09999999999999999167 ) ;
#118913=EDGE_LOOP ( 'NONE', ( #36947, #3015, #77188, #117389 ) ) ;
#118914=DIRECTION ( 'NONE',  ( -0.000000000000000000, -1.000000000000000000, -0.000000000000000000 ) ) ;
#118915=ADVANCED_FACE ( 'NONE', ( #82724 ), #53796, .T. ) ;
#118916=AXIS2_PLACEMENT_3D ( 'NONE', #96014, #27263, #26629 ) ;
#118917=EDGE_CURVE ( 'NONE', #84838, #29011, #44068, .T. ) ;
#118918=DIRECTION ( 'NONE',  ( -0.000000000000000000, 1.000000000000000000, -0.000000000000000000 ) ) ;
#118919=CARTESIAN_POINT ( 'NONE',  ( 12.49999999999990408, 2.500000000000000000, -3.537306695894649966 ) ) ;
#118920=ORIENTED_EDGE ( 'NONE', *, *, #15535, .T. ) ;
#118921=AXIS2_PLACEMENT_3D ( 'NONE', #43632, #45559, #95933 ) ;
#118922=ORIENTED_EDGE ( 'NONE', *, *, #109861, .T. ) ;
#118923=ADVANCED_FACE ( 'NONE', ( #2852 ), #83360, .T. ) ;
#118924=CARTESIAN_POINT ( 'NONE',  ( -3.150000000000032330, 2.500000000000000000, -6.048780366869526581 ) ) ;
#118925=CIRCLE ( 'NONE', #79231, 0.1000000000000002554 ) ;
#118926=ADVANCED_FACE ( 'NONE', ( #70952 ), #110235, .T. ) ;
#118927=ORIENTED_EDGE ( 'NONE', *, *, #47184, .T. ) ;
#118928=ORIENTED_EDGE ( 'NONE', *, *, #32335, .T. ) ;
#118929=ORIENTED_EDGE ( 'NONE', *, *, #59937, .T. ) ;
#118930=CARTESIAN_POINT ( 'NONE',  ( 5.649999999999934630, 12.50000000000000000, 6.148780366869520897 ) ) ;
#118931=DIRECTION ( 'NONE',  ( 0.000000000000000000, -0.000000000000000000, 1.000000000000000000 ) ) ;
#118932=FACE_OUTER_BOUND ( 'NONE', #69233, .T. ) ;
#118933=DIRECTION ( 'NONE',  ( 0.000000000000000000, 0.000000000000000000, -1.000000000000000000 ) ) ;
#118934=AXIS2_PLACEMENT_3D ( 'NONE', #5492, #122236, #36280 ) ;
#118935=EDGE_LOOP ( 'NONE', ( #73446, #54734, #74635, #107913 ) ) ;
#118936=CARTESIAN_POINT ( 'NONE',  ( 0.6499999999999543920, 2.500000000000000000, 6.841600689897072485 ) ) ;
#118937=ORIENTED_EDGE ( 'NONE', *, *, #91218, .T. ) ;
#118938=DIRECTION ( 'NONE',  ( -0.000000000000000000, 1.000000000000000000, -0.000000000000000000 ) ) ;
#118939=CARTESIAN_POINT ( 'NONE',  ( 18.87984495337894586, 0.5408627091909939955, 4.542689527608590794 ) ) ;
#118940=DIRECTION ( 'NONE',  ( 0.000000000000000000, 1.000000000000000000, 0.000000000000000000 ) ) ;
#118941=DIRECTION ( 'NONE',  ( -0.000000000000000000, 1.000000000000000000, -0.000000000000000000 ) ) ;
#118942=ORIENTED_EDGE ( 'NONE', *, *, #35828, .F. ) ;
#118943=AXIS2_PLACEMENT_3D ( 'NONE', #58051, #129389, #88109 ) ;
#118944=VERTEX_POINT ( 'NONE', #101054 ) ;
#118946=EDGE_LOOP ( 'NONE', ( #33135, #117269, #48351, #127415 ) ) ;
#118947=ORIENTED_EDGE ( 'NONE', *, *, #36885, .F. ) ;
#118948=DIRECTION ( 'NONE',  ( 0.000000000000000000, 0.000000000000000000, -1.000000000000000000 ) ) ;
#118949=DIRECTION ( 'NONE',  ( 0.000000000000000000, 0.000000000000000000, 1.000000000000000000 ) ) ;
#118950=DIRECTION ( 'NONE',  ( 0.000000000000000000, 0.000000000000000000, 1.000000000000000000 ) ) ;
#118951=FACE_BOUND ( 'NONE', #35574, .T. ) ;
#118952=LINE ( 'NONE', #109112, #110029 ) ;
#118954=AXIS2_PLACEMENT_3D ( 'NONE', #87309, #105679, #6790 ) ;
#118955=DIRECTION ( 'NONE',  ( 0.000000000000000000, 0.000000000000000000, 1.000000000000000000 ) ) ;
#118956=CARTESIAN_POINT ( 'NONE',  ( -9.800000000000004263, 12.50000000000000000, -0.2813168883297409439 ) ) ;
#118957=AXIS2_PLACEMENT_3D ( 'NONE', #93990, #63241, #73691 ) ;
#118958=CARTESIAN_POINT ( 'NONE',  ( 3.749999999999978684, 2.500000000000000000, -6.395190528383301931 ) ) ;
#118959=DIRECTION ( 'NONE',  ( 0.000000000000000000, 0.000000000000000000, -1.000000000000000000 ) ) ;
#118960=CIRCLE ( 'NONE', #62545, 0.1000000000000002554 ) ;
#118961=DIRECTION ( 'NONE',  ( 0.000000000000000000, 1.000000000000000000, 0.000000000000000000 ) ) ;
#118962=EDGE_CURVE ( 'NONE', #65442, #123620, #47549, .T. ) ;
#118963=LINE ( 'NONE', #61993, #76523 ) ;
#118964=AXIS2_PLACEMENT_3D ( 'NONE', #108754, #78682, #98291 ) ;
#118965=ORIENTED_EDGE ( 'NONE', *, *, #105846, .T. ) ;
#118966=ORIENTED_EDGE ( 'NONE', *, *, #53732, .F. ) ;
#118967=VERTEX_POINT ( 'NONE', #51969 ) ;
#118968=VERTEX_POINT ( 'NONE', #103641 ) ;
#118969=ADVANCED_FACE ( 'NONE', ( #73516 ), #9889, .T. ) ;
#118970=CARTESIAN_POINT ( 'NONE',  ( 12.09999999999990195, 12.50000000000000000, 0.6928203230275494784 ) ) ;
#118971=AXIS2_PLACEMENT_3D ( 'NONE', #116235, #68428, #18686 ) ;
#118972=CARTESIAN_POINT ( 'NONE',  ( -5.650000000000023448, 2.500000000000000000, -6.248780366869526759 ) ) ;
#118973=EDGE_CURVE ( 'NONE', #78706, #37294, #83058, .T. ) ;
#118974=FACE_BOUND ( 'NONE', #45362, .T. ) ;
#118975=CARTESIAN_POINT ( 'NONE',  ( -3.750000000000027534, 12.50000000000000000, 2.792790559304612064 ) ) ;
#118976=AXIS2_PLACEMENT_3D ( 'NONE', #83008, #65266, #3788 ) ;
#118977=CIRCLE ( 'NONE', #70867, 0.1000000000000000472 ) ;
#118979=DIRECTION ( 'NONE',  ( 0.000000000000000000, 0.000000000000000000, 1.000000000000000000 ) ) ;
#118980=LINE ( 'NONE', #60716, #118408 ) ;
#118981=ADVANCED_FACE ( 'NONE', ( #71594 ), #18286, .T. ) ;
#118982=DIRECTION ( 'NONE',  ( 0.000000000000000000, 1.000000000000000000, 0.000000000000000000 ) ) ;
#118983=LINE ( 'NONE', #32410, #70881 ) ;
#118984=DIRECTION ( 'NONE',  ( -4.274815082592931898E-19, -0.9999939076577903929, -0.003490651415223739937 ) ) ;
#118985=VERTEX_POINT ( 'NONE', #111514 ) ;
#118986=FACE_OUTER_BOUND ( 'NONE', #35629, .T. ) ;
#118987=ORIENTED_EDGE ( 'NONE', *, *, #28005, .T. ) ;
#118988=ORIENTED_EDGE ( 'NONE', *, *, #117975, .T. ) ;
#118989=AXIS2_PLACEMENT_3D ( 'NONE', #46709, #125893, #94505 ) ;
#118990=CARTESIAN_POINT ( 'NONE',  ( -12.89999999999999147, 2.500000000000000000, 4.330127018922196314 ) ) ;
#118991=DIRECTION ( 'NONE',  ( 0.000000000000000000, 0.000000000000000000, 1.000000000000000000 ) ) ;
#118992=ORIENTED_EDGE ( 'NONE', *, *, #70109, .T. ) ;
#118993=CIRCLE ( 'NONE', #47909, 0.1000000000000002554 ) ;
#118994=CARTESIAN_POINT ( 'NONE',  ( -1.050000000000037792, 2.500000000000000000, 6.248780366869520542 ) ) ;
#118995=CONICAL_SURFACE ( 'NONE', #114780, 0.1000000000000002554, 0.003490658503988666988 ) ;
#118996=CARTESIAN_POINT ( 'NONE',  ( 13.29999999999990301, 2.500000000000000000, 4.330127018922196314 ) ) ;
#118997=EDGE_LOOP ( 'NONE', ( #51976, #54449, #30974, #47349 ) ) ;
#118998=FACE_OUTER_BOUND ( 'NONE', #58386, .T. ) ;
#118999=ORIENTED_EDGE ( 'NONE', *, *, #11406, .F. ) ;
#119000=CARTESIAN_POINT ( 'NONE',  ( 13.09999999999990195, 12.50000000000000000, -4.676537180435978769 ) ) ;
#119001=AXIS2_PLACEMENT_3D ( 'NONE', #71573, #3481, #112801 ) ;
#119002=EDGE_LOOP ( 'NONE', ( #11552, #92339 ) ) ;
#119004=FACE_BOUND ( 'NONE', #37023, .T. ) ;
#119005=CIRCLE ( 'NONE', #114794, 0.09999999999999982514 ) ;
#119006=EDGE_CURVE ( 'NONE', #80728, #120532, #120700, .T. ) ;
#119007=CONICAL_SURFACE ( 'NONE', #62589, 0.1000000000000002554, 0.003490658503988666988 ) ;
#119008=ORIENTED_EDGE ( 'NONE', *, *, #53376, .F. ) ;
#119009=DIRECTION ( 'NONE',  ( 0.000000000000000000, 1.000000000000000000, 0.000000000000000000 ) ) ;
#119010=EDGE_LOOP ( 'NONE', ( #120958, #88082 ) ) ;
#119011=DIRECTION ( 'NONE',  ( -0.000000000000000000, 1.000000000000000000, -0.000000000000000000 ) ) ;
#119012=CARTESIAN_POINT ( 'NONE',  ( -2.100000000000034284, 2.500000000000000000, -0.1000000000000023925 ) ) ;
#119014=DIRECTION ( 'NONE',  ( 0.000000000000000000, 1.000000000000000000, 0.000000000000000000 ) ) ;
#119015=DIRECTION ( 'NONE',  ( -4.274815082592931898E-19, -0.9999939076577903929, -0.003490651415223739937 ) ) ;
#119016=ADVANCED_FACE ( 'NONE', ( #82050 ), #99777, .T. ) ;
#119017=EDGE_CURVE ( 'NONE', #75397, #95423, #23136, .T. ) ;
#119018=CARTESIAN_POINT ( 'NONE',  ( 12.89999999999990266, 12.50000000000000000, 5.022947341949748790 ) ) ;
#119019=AXIS2_PLACEMENT_3D ( 'NONE', #114766, #44096, #93214 ) ;
#119021=EDGE_LOOP ( 'NONE', ( #19674, #56823, #37560, #28432 ) ) ;
#119022=ORIENTED_EDGE ( 'NONE', *, *, #2226, .F. ) ;
#119023=AXIS2_PLACEMENT_3D ( 'NONE', #108911, #41510, #31046 ) ;
#119024=ORIENTED_EDGE ( 'NONE', *, *, #104631, .T. ) ;
#119025=DIRECTION ( 'NONE',  ( 0.000000000000000000, 1.000000000000000000, 0.000000000000000000 ) ) ;
#119026=CONICAL_SURFACE ( 'NONE', #108559, 0.1000000000000002554, 0.003490658503988666988 ) ;
#119027=DIRECTION ( 'NONE',  ( 0.000000000000000000, 1.000000000000000000, 0.000000000000000000 ) ) ;
#119028=EDGE_CURVE ( 'NONE', #78573, #47526, #64258, .T. ) ;
#119029=CARTESIAN_POINT ( 'NONE',  ( 12.94999999999989981, 12.50000000000000000, -2.165063509461101710 ) ) ;
#119030=ORIENTED_EDGE ( 'NONE', *, *, #110394, .F. ) ;
#119031=VERTEX_POINT ( 'NONE', #114099 ) ;
#119032=EDGE_LOOP ( 'NONE', ( #65952, #108971, #66483, #115740 ) ) ;
#119033=ADVANCED_FACE ( 'NONE', ( #34916 ), #46648, .T. ) ;
#119034=DIRECTION ( 'NONE',  ( 0.000000000000000000, 0.000000000000000000, 1.000000000000000000 ) ) ;
#119035=CARTESIAN_POINT ( 'NONE',  ( -13.09999999999999254, 2.500000000000000000, -0.3464101615137741286 ) ) ;
#119037=EDGE_CURVE ( 'NONE', #84136, #101321, #55181, .T. ) ;
#119038=DIRECTION ( 'NONE',  ( -4.274815082592931898E-19, -0.9999939076577903929, -0.003490651415223739937 ) ) ;
#119040=LINE ( 'NONE', #535, #21465 ) ;
#119041=DIRECTION ( 'NONE',  ( 0.000000000000000000, 1.000000000000000000, 0.000000000000000000 ) ) ;
#119042=VECTOR ( 'NONE', #25801, 1000.000000000000000 ) ;
#119043=DIRECTION ( 'NONE',  ( 0.000000000000000000, 0.000000000000000000, 1.000000000000000000 ) ) ;
#119044=EDGE_CURVE ( 'NONE', #38154, #124518, #74176, .T. ) ;
#119045=CARTESIAN_POINT ( 'NONE',  ( 7.899999999999921307, 2.500000000000000000, -0.1000000000000023925 ) ) ;
#119046=EDGE_CURVE ( 'NONE', #60634, #114454, #104902, .T. ) ;
#119047=ORIENTED_EDGE ( 'NONE', *, *, #126734, .F. ) ;
#119048=ORIENTED_EDGE ( 'NONE', *, *, #8366, .F. ) ;
#119049=CARTESIAN_POINT ( 'NONE',  ( 2.099999999999949463, 2.500000000000000000, 0.5928203230275495006 ) ) ;
#119050=CARTESIAN_POINT ( 'NONE',  ( 7.499999999999927169, 2.500000000000000000, -5.022947341949754119 ) ) ;
#119051=ORIENTED_EDGE ( 'NONE', *, *, #89241, .F. ) ;
#119052=EDGE_LOOP ( 'NONE', ( #37171, #17952, #49384, #33686 ) ) ;
#119055=CARTESIAN_POINT ( 'NONE',  ( -11.25000000000000000, 2.500000000000000000, -2.857883832488649745 ) ) ;
#119056=CIRCLE ( 'NONE', #54211, 0.06509327318403745899 ) ;
#119057=DIRECTION ( 'NONE',  ( 0.000000000000000000, 1.000000000000000000, 0.000000000000000000 ) ) ;
#119058=CARTESIAN_POINT ( 'NONE',  ( 1.649999999999951505, 2.500000000000000000, 1.572243186433545548 ) ) ;
#119059=DIRECTION ( 'NONE',  ( 0.000000000000000000, -0.000000000000000000, 1.000000000000000000 ) ) ;
#119060=CARTESIAN_POINT ( 'NONE',  ( -10.65000000000000391, 2.500000000000000000, -2.611473670974873595 ) ) ;
#119061=DIRECTION ( 'NONE',  ( 0.000000000000000000, 0.000000000000000000, 1.000000000000000000 ) ) ;
#119062=AXIS2_PLACEMENT_3D ( 'NONE', #28393, #67652, #77479 ) ;
#119063=FACE_OUTER_BOUND ( 'NONE', #68820, .T. ) ;
#119064=VERTEX_POINT ( 'NONE', #66913 ) ;
#119065=CIRCLE ( 'NONE', #6174, 0.1000000000000002554 ) ;
#119066=VECTOR ( 'NONE', #20117, 1000.000000000000000 ) ;
#119067=ORIENTED_EDGE ( 'NONE', *, *, #91991, .F. ) ;
#119068=CIRCLE ( 'NONE', #52171, 0.06509327318403745899 ) ;
#119069=ORIENTED_EDGE ( 'NONE', *, *, #73607, .T. ) ;
#119070=ORIENTED_EDGE ( 'NONE', *, *, #28607, .F. ) ;
#119071=DIRECTION ( 'NONE',  ( 0.000000000000000000, 0.000000000000000000, 1.000000000000000000 ) ) ;
#119072=DIRECTION ( 'NONE',  ( 0.000000000000000000, 0.000000000000000000, -1.000000000000000000 ) ) ;
#119073=AXIS2_PLACEMENT_3D ( 'NONE', #116300, #46280, #65919 ) ;
#119074=CIRCLE ( 'NONE', #116991, 0.06509327318403745899 ) ;
#119075=ORIENTED_EDGE ( 'NONE', *, *, #30600, .F. ) ;
#119076=CARTESIAN_POINT ( 'NONE',  ( 1.849999999999950129, 12.50000000000000000, -6.841600689897078702 ) ) ;
#119077=EDGE_CURVE ( 'NONE', #100531, #115634, #104279, .T. ) ;
#119078=DIRECTION ( 'NONE',  ( 0.000000000000000000, 0.000000000000000000, 1.000000000000000000 ) ) ;
#119079=ADVANCED_FACE ( 'NONE', ( #116025 ), #85191, .T. ) ;
#119080=CARTESIAN_POINT ( 'NONE',  ( -10.85000000000000142, 12.50000000000000000, 6.495190528383297135 ) ) ;
#119081=DIRECTION ( 'NONE',  ( -4.274815082592931898E-19, -0.9999939076577903929, -0.003490651415223739937 ) ) ;
#119082=ORIENTED_EDGE ( 'NONE', *, *, #117179, .T. ) ;
#119084=PLANE ( 'NONE',  #87492 ) ;
#119085=ORIENTED_EDGE ( 'NONE', *, *, #26593, .T. ) ;
#119087=VERTEX_POINT ( 'NONE', #54516 ) ;
#119088=CIRCLE ( 'NONE', #38749, 0.1000000000000000056 ) ;
#119089=ORIENTED_EDGE ( 'NONE', *, *, #78075, .F. ) ;
#119090=DIRECTION ( 'NONE',  ( -0.000000000000000000, -1.000000000000000000, -0.000000000000000000 ) ) ;
#119091=DIRECTION ( 'NONE',  ( 0.000000000000000000, -0.000000000000000000, 1.000000000000000000 ) ) ;
#119092=CARTESIAN_POINT ( 'NONE',  ( -7.300000000000014921, 2.500000000000000000, 4.676537180435972552 ) ) ;
#119093=CIRCLE ( 'NONE', #58467, 0.09999999999999999167 ) ;
#119094=CIRCLE ( 'NONE', #96099, 0.09999999999999982514 ) ;
#119095=ORIENTED_EDGE ( 'NONE', *, *, #116429, .T. ) ;
#119096=LINE ( 'NONE', #69332, #45512 ) ;
#119097=DIRECTION ( 'NONE',  ( 0.000000000000000000, 0.000000000000000000, -1.000000000000000000 ) ) ;
#119098=DIRECTION ( 'NONE',  ( 0.000000000000000000, 1.000000000000000000, 0.000000000000000000 ) ) ;
#119099=DIRECTION ( 'NONE',  ( 0.000000000000000000, 0.000000000000000000, -1.000000000000000000 ) ) ;
#119100=AXIS2_PLACEMENT_3D ( 'NONE', #113273, #112643, #123104 ) ;
#119101=CIRCLE ( 'NONE', #33440, 0.06509327318403745899 ) ;
#119102=ORIENTED_EDGE ( 'NONE', *, *, #92127, .F. ) ;
#119103=DIRECTION ( 'NONE',  ( 0.000000000000000000, 0.000000000000000000, -1.000000000000000000 ) ) ;
#119104=EDGE_LOOP ( 'NONE', ( #83104, #31659 ) ) ;
#119105=ORIENTED_EDGE ( 'NONE', *, *, #4452, .T. ) ;
#119106=CARTESIAN_POINT ( 'NONE',  ( -0.6500000000000394351, 2.500000000000000000, 6.841600689897072485 ) ) ;
#119107=DIRECTION ( 'NONE',  ( 0.000000000000000000, 0.000000000000000000, -1.000000000000000000 ) ) ;
#119108=FACE_BOUND ( 'NONE', #19192, .T. ) ;
#119109=CIRCLE ( 'NONE', #89855, 0.09999999999999982514 ) ;
#119110=LINE ( 'NONE', #68067, #7510 ) ;
#119111=PLANE ( 'NONE',  #107126 ) ;
#119112=DIRECTION ( 'NONE',  ( -0.000000000000000000, 1.000000000000000000, -0.000000000000000000 ) ) ;
#119113=CIRCLE ( 'NONE', #108641, 0.1000000000000002554 ) ;
#119114=EDGE_CURVE ( 'NONE', #42431, #105649, #76753, .T. ) ;
#119115=AXIS2_PLACEMENT_3D ( 'NONE', #51188, #72112, #112677 ) ;
#119116=VERTEX_POINT ( 'NONE', #4763 ) ;
#119117=CARTESIAN_POINT ( 'NONE',  ( -0.6000000000000323963, 2.500000000000000000, -0.3464101615137759604 ) ) ;
#119118=CARTESIAN_POINT ( 'NONE',  ( 11.64999999999990798, 12.50000000000000000, -2.792790559304616504 ) ) ;
#119119=DIRECTION ( 'NONE',  ( -0.000000000000000000, -1.000000000000000000, -0.000000000000000000 ) ) ;
#119120=CARTESIAN_POINT ( 'NONE',  ( 0.8499999999999557909, 2.500000000000000000, -7.088010851410853519 ) ) ;
#119121=VERTEX_POINT ( 'NONE', #5420 ) ;
#119122=AXIS2_PLACEMENT_3D ( 'NONE', #112022, #122490, #63569 ) ;
#119123=ADVANCED_FACE ( 'NONE', ( #44725 ), #91448, .T. ) ;
#119124=FACE_OUTER_BOUND ( 'NONE', #93333, .T. ) ;
#119125=DIRECTION ( 'NONE',  ( 0.000000000000000000, 0.000000000000000000, -1.000000000000000000 ) ) ;
#119126=AXIS2_PLACEMENT_3D ( 'NONE', #43376, #42076, #83295 ) ;
#119128=ORIENTED_EDGE ( 'NONE', *, *, #125840, .F. ) ;
#119129=ADVANCED_FACE ( 'NONE', ( #27013 ), #5746, .T. ) ;
#119130=DIRECTION ( 'NONE',  ( 0.000000000000000000, 0.000000000000000000, 1.000000000000000000 ) ) ;
#119131=CARTESIAN_POINT ( 'NONE',  ( -5.000000000000023093, 12.50000000000000000, 5.022947341949748790 ) ) ;
#119132=EDGE_CURVE ( 'NONE', #74569, #23572, #114734, .T. ) ;
#119133=FACE_BOUND ( 'NONE', #85883, .T. ) ;
#119134=CARTESIAN_POINT ( 'NONE',  ( 5.199999999999935341, 12.50000000000000000, -3.983716857408426293 ) ) ;
#119135=DIRECTION ( 'NONE',  ( -0.000000000000000000, 1.000000000000000000, -0.000000000000000000 ) ) ;
#119136=ORIENTED_EDGE ( 'NONE', *, *, #7306, .T. ) ;
#119137=CARTESIAN_POINT ( 'NONE',  ( -9.350000000000006750, 2.500000000000000000, -2.611473670974877592 ) ) ;
#119138=ADVANCED_FACE ( 'NONE', ( #75449 ), #30919, .T. ) ;
#119140=ORIENTED_EDGE ( 'NONE', *, *, #106639, .T. ) ;
#119141=CARTESIAN_POINT ( 'NONE',  ( 13.54999999999989591, 2.500000000000000000, -1.718653347947326049 ) ) ;
#119142=CARTESIAN_POINT ( 'NONE',  ( -9.200000000000006395, 2.500000000000000000, -2.385244779468109755E-15 ) ) ;
#119143=PLANE ( 'NONE',  #121720 ) ;
#119144=AXIS2_PLACEMENT_3D ( 'NONE', #10357, #109857, #40489 ) ;
#119145=CARTESIAN_POINT ( 'NONE',  ( -6.650000000000014566, 2.500000000000000000, 2.265063509461097357 ) ) ;
#119146=EDGE_LOOP ( 'NONE', ( #86223, #106602 ) ) ;
#119147=CIRCLE ( 'NONE', #79460, 0.09999999999999982514 ) ;
#119148=CIRCLE ( 'NONE', #106532, 0.09999999999999982514 ) ;
#119149=CARTESIAN_POINT ( 'NONE',  ( -0.4000000000000339950, 12.50000000000000000, 0.7579135962115892688 ) ) ;
#119150=DIRECTION ( 'NONE',  ( 0.000000000000000000, 1.000000000000000000, 0.000000000000000000 ) ) ;
#119151=CARTESIAN_POINT ( 'NONE',  ( 16.56034315062901641, 0.8287392047036494791, -6.090234455234604383 ) ) ;
#119152=VERTEX_POINT ( 'NONE', #105570 ) ;
#119153=EDGE_LOOP ( 'NONE', ( #30731, #90891 ) ) ;
#119154=DIRECTION ( 'NONE',  ( 0.000000000000000000, 1.000000000000000000, 0.000000000000000000 ) ) ;
#119155=ORIENTED_EDGE ( 'NONE', *, *, #118585, .T. ) ;
#119156=LINE ( 'NONE', #79249, #32362 ) ;
#119157=CIRCLE ( 'NONE', #77398, 0.1000000000000002554 ) ;
#119158=VECTOR ( 'NONE', #89014, 1000.000000000000000 ) ;
#119159=CARTESIAN_POINT ( 'NONE',  ( -8.150000000000009237, 2.500000000000000000, 6.741600689897071952 ) ) ;
#119160=EDGE_CURVE ( 'NONE', #61030, #73196, #112484, .T. ) ;
#119161=CARTESIAN_POINT ( 'NONE',  ( -11.64999999999999680, 2.500000000000000000, 7.188010851410848723 ) ) ;
#119162=VERTEX_POINT ( 'NONE', #106214 ) ;
#119163=CARTESIAN_POINT ( 'NONE',  ( -5.850000000000019185, 12.50000000000000000, 2.230156782645134950 ) ) ;
#119164=CARTESIAN_POINT ( 'NONE',  ( -3.150000000000029221, 2.500000000000000000, 2.411473670974873862 ) ) ;
#119165=LINE ( 'NONE', #89070, #94554 ) ;
#119166=DIRECTION ( 'NONE',  ( 0.000000000000000000, 0.000000000000000000, 1.000000000000000000 ) ) ;
#119167=CARTESIAN_POINT ( 'NONE',  ( 3.749999999999938716, 2.500000000000000000, 7.088010851410848190 ) ) ;
#119169=DIRECTION ( 'NONE',  ( 0.000000000000000000, 0.000000000000000000, 1.000000000000000000 ) ) ;
#119170=EDGE_CURVE ( 'NONE', #23744, #61622, #35132, .T. ) ;
#119171=ORIENTED_EDGE ( 'NONE', *, *, #62134, .T. ) ;
#119172=ORIENTED_EDGE ( 'NONE', *, *, #50626, .T. ) ;
#119173=DIRECTION ( 'NONE',  ( -0.000000000000000000, 1.000000000000000000, -0.000000000000000000 ) ) ;
#119174=EDGE_LOOP ( 'NONE', ( #41382, #124579, #62661, #17074 ) ) ;
#119176=EDGE_CURVE ( 'NONE', #101758, #17235, #3709, .T. ) ;
#119177=ORIENTED_EDGE ( 'NONE', *, *, #28699, .T. ) ;
#119178=ORIENTED_EDGE ( 'NONE', *, *, #110627, .T. ) ;
#119179=ADVANCED_FACE ( 'NONE', ( #127152 ), #114516, .T. ) ;
#119180=ORIENTED_EDGE ( 'NONE', *, *, #33888, .F. ) ;
#119181=EDGE_CURVE ( 'NONE', #31716, #31853, #39343, .T. ) ;
#119182=CARTESIAN_POINT ( 'NONE',  ( 17.50000000000000000, 2.083333333333335258, -3.999999999999996447 ) ) ;
#119183=EDGE_CURVE ( 'NONE', #97290, #85218, #120787, .T. ) ;
#119184=CIRCLE ( 'NONE', #39783, 0.06509327318403745899 ) ;
#119185=CARTESIAN_POINT ( 'NONE',  ( -2.300000000000033573, 12.50000000000000000, -3.918623584224389056 ) ) ;
#119186=CIRCLE ( 'NONE', #43895, 0.06509327318403745899 ) ;
#119187=DIRECTION ( 'NONE',  ( 0.000000000000000000, 0.000000000000000000, -1.000000000000000000 ) ) ;
#119189=EDGE_CURVE ( 'NONE', #113481, #86732, #20414, .T. ) ;
#119190=PLANE ( 'NONE',  #51420 ) ;
#119191=DIRECTION ( 'NONE',  ( -0.000000000000000000, 1.000000000000000000, -0.000000000000000000 ) ) ;
#119192=CARTESIAN_POINT ( 'NONE',  ( -3.150000000000030109, 12.50000000000000000, -2.511473670974877948 ) ) ;
#119193=CARTESIAN_POINT ( 'NONE',  ( 5.399999999999936406, 12.50000000000000000, -5.022947341949754119 ) ) ;
#119194=DIRECTION ( 'NONE',  ( 0.000000000000000000, 0.000000000000000000, -1.000000000000000000 ) ) ;
#119195=DIRECTION ( 'NONE',  ( -0.000000000000000000, 1.000000000000000000, -0.000000000000000000 ) ) ;
#119196=AXIS2_PLACEMENT_3D ( 'NONE', #14279, #75152, #34606 ) ;
#119197=EDGE_CURVE ( 'NONE', #56994, #125139, #108268, .T. ) ;
#119198=ORIENTED_EDGE ( 'NONE', *, *, #764, .T. ) ;
#119199=ADVANCED_FACE ( 'NONE', ( #59051 ), #78039, .T. ) ;
#119200=EDGE_LOOP ( 'NONE', ( #66044, #11337, #23895, #19471 ) ) ;
#119201=CARTESIAN_POINT ( 'NONE',  ( -2.100000000000033840, 2.500000000000000000, 3.637306695894644726 ) ) ;
#119202=ORIENTED_EDGE ( 'NONE', *, *, #58363, .F. ) ;
#119204=DIRECTION ( 'NONE',  ( -4.274815082592931898E-19, -0.9999939076577903929, -0.003490651415223739937 ) ) ;
#119205=AXIS2_PLACEMENT_3D ( 'NONE', #60707, #53468, #90800 ) ;
#119206=VECTOR ( 'NONE', #64824, 1000.000000000000000 ) ;
#119207=DIRECTION ( 'NONE',  ( 0.000000000000000000, -0.000000000000000000, 1.000000000000000000 ) ) ;
#119208=CIRCLE ( 'NONE', #66951, 0.1000000000000002554 ) ;
#119209=CARTESIAN_POINT ( 'NONE',  ( -0.8500000000000382805, 2.500000000000000000, -1.372243186433550033 ) ) ;
#119210=FACE_OUTER_BOUND ( 'NONE', #88144, .T. ) ;
#119211=LINE ( 'NONE', #60315, #71886 ) ;
#119212=ORIENTED_EDGE ( 'NONE', *, *, #127895, .F. ) ;
#119213=CIRCLE ( 'NONE', #104624, 0.1000000000000002554 ) ;
#119214=ORIENTED_EDGE ( 'NONE', *, *, #115934, .T. ) ;
#119215=CARTESIAN_POINT ( 'NONE',  ( 11.44999999999990514, 12.50000000000000000, -6.148780366869526226 ) ) ;
#119216=ORIENTED_EDGE ( 'NONE', *, *, #85012, .T. ) ;
#119217=DIRECTION ( 'NONE',  ( -0.000000000000000000, 1.000000000000000000, -0.000000000000000000 ) ) ;
#119218=AXIS2_PLACEMENT_3D ( 'NONE', #47170, #37983, #117162 ) ;
#119219=ORIENTED_EDGE ( 'NONE', *, *, #50167, .F. ) ;
#119220=ORIENTED_EDGE ( 'NONE', *, *, #23708, .F. ) ;
#119221=CARTESIAN_POINT ( 'NONE',  ( 10.44999999999991047, 12.50000000000000000, -6.495190528383302464 ) ) ;
#119222=CARTESIAN_POINT ( 'NONE',  ( 10.84999999999991260, 2.500000000000000000, 5.902370205355745192 ) ) ;
#119223=LINE ( 'NONE', #88, #84297 ) ;
#119224=EDGE_CURVE ( 'NONE', #109349, #102868, #89144, .T. ) ;
#119225=DIRECTION ( 'NONE',  ( -0.000000000000000000, -1.000000000000000000, -0.000000000000000000 ) ) ;
#119226=CARTESIAN_POINT ( 'NONE',  ( 7.099999999999928590, 2.500000000000000000, -5.122947341949753763 ) ) ;
#119227=EDGE_LOOP ( 'NONE', ( #67281, #98255 ) ) ;
#119228=CARTESIAN_POINT ( 'NONE',  ( -13.29999999999998828, 2.500000000000000000, 4.330127018922196314 ) ) ;
#119229=DIRECTION ( 'NONE',  ( -0.000000000000000000, 1.000000000000000000, -0.000000000000000000 ) ) ;
#119230=CARTESIAN_POINT ( 'NONE',  ( -9.600000000000006750, 12.50000000000000000, 5.022947341949748790 ) ) ;
#119231=CARTESIAN_POINT ( 'NONE',  ( 3.349999999999945466, 2.500000000000000000, -6.595190528383302109 ) ) ;
#119232=DIRECTION ( 'NONE',  ( -0.000000000000000000, -1.000000000000000000, -0.000000000000000000 ) ) ;
#119233=EDGE_CURVE ( 'NONE', #17511, #111104, #93602, .T. ) ;
#119235=ORIENTED_EDGE ( 'NONE', *, *, #41302, .F. ) ;
#119236=FACE_OUTER_BOUND ( 'NONE', #75344, .T. ) ;
#119237=AXIS2_PLACEMENT_3D ( 'NONE', #11645, #32611, #72514 ) ;
#119238=ORIENTED_EDGE ( 'NONE', *, *, #48014, .T. ) ;
#119239=DIRECTION ( 'NONE',  ( 0.000000000000000000, 0.000000000000000000, 1.000000000000000000 ) ) ;
#119240=FACE_OUTER_BOUND ( 'NONE', #92753, .T. ) ;
#119241=AXIS2_PLACEMENT_3D ( 'NONE', #85275, #113449, #72257 ) ;
#119242=VECTOR ( 'NONE', #121370, 1000.000000000000000 ) ;
#119243=VERTEX_POINT ( 'NONE', #9298 ) ;
#119244=DIRECTION ( 'NONE',  ( 0.000000000000000000, 0.000000000000000000, 1.000000000000000000 ) ) ;
#119246=DIRECTION ( 'NONE',  ( 0.000000000000000000, 0.000000000000000000, 1.000000000000000000 ) ) ;
#119247=CARTESIAN_POINT ( 'NONE',  ( -7.300000000000014921, 2.500000000000000000, 4.676537180435972552 ) ) ;
#119248=PLANE ( 'NONE',  #68688 ) ;
#119249=ORIENTED_EDGE ( 'NONE', *, *, #30969, .T. ) ;
#119250=CARTESIAN_POINT ( 'NONE',  ( 59.74179236529985815, 3.401974343112436738, -5.439312642699807299 ) ) ;
#119251=CARTESIAN_POINT ( 'NONE',  ( -12.49999999999995737, 12.50000000000000000, 4.330127018922196314 ) ) ;
#119252=DIRECTION ( 'NONE',  ( -0.000000000000000000, -1.000000000000000000, -0.000000000000000000 ) ) ;
#119253=ADVANCED_FACE ( 'NONE', ( #17817 ), #72762, .T. ) ;
#119254=EDGE_LOOP ( 'NONE', ( #128879, #123522, #4475, #95439 ) ) ;
#119255=DIRECTION ( 'NONE',  ( -0.000000000000000000, 1.000000000000000000, -0.000000000000000000 ) ) ;
#119256=ORIENTED_EDGE ( 'NONE', *, *, #78108, .T. ) ;
#119257=PLANE ( 'NONE',  #121168 ) ;
#119258=CARTESIAN_POINT ( 'NONE',  ( 8.749999999999921840, 12.50000000000000000, 2.792790559304612064 ) ) ;
#119259=CARTESIAN_POINT ( 'NONE',  ( 11.04999999999990656, 12.50000000000000000, -6.148780366869526226 ) ) ;
#119260=ORIENTED_EDGE ( 'NONE', *, *, #129246, .F. ) ;
#119261=VECTOR ( 'NONE', #98940, 1000.000000000000000 ) ;
#119262=EDGE_CURVE ( 'NONE', #44544, #27907, #87325, .T. ) ;
#119263=CARTESIAN_POINT ( 'NONE',  ( 6.049999999999932321, 12.50000000000000000, 1.818653347947321475 ) ) ;
#119264=VECTOR ( 'NONE', #64619, 1000.000000000000000 ) ;
#119266=EDGE_CURVE ( 'NONE', #43427, #88605, #27627, .T. ) ;
#119267=VERTEX_POINT ( 'NONE', #68208 ) ;
#119268=EDGE_CURVE ( 'NONE', #123245, #59339, #68548, .T. ) ;
#119269=DIRECTION ( 'NONE',  ( 0.000000000000000000, 0.000000000000000000, 1.000000000000000000 ) ) ;
#119270=ADVANCED_FACE ( 'NONE', ( #49887 ), #5846, .T. ) ;
#119271=ORIENTED_EDGE ( 'NONE', *, *, #20753, .F. ) ;
#119272=CIRCLE ( 'NONE', #92083, 0.1000000000000000472 ) ;
#119273=FACE_OUTER_BOUND ( 'NONE', #25278, .T. ) ;
#119274=ORIENTED_EDGE ( 'NONE', *, *, #29805, .F. ) ;
#119275=DIRECTION ( 'NONE',  ( 0.000000000000000000, -0.9999939076577903929, 0.003490651415223739937 ) ) ;
#119276=CARTESIAN_POINT ( 'NONE',  ( 6.899999999999926636, 12.50000000000000000, -0.2813168883297408329 ) ) ;
#119277=ADVANCED_FACE ( 'NONE', ( #59716 ), #57766, .T. ) ;
#119278=EDGE_LOOP ( 'NONE', ( #70608, #61769, #40707, #21238 ) ) ;
#119279=ORIENTED_EDGE ( 'NONE', *, *, #10663, .F. ) ;
#119280=EDGE_CURVE ( 'NONE', #61052, #95146, #102013, .T. ) ;
#119281=CARTESIAN_POINT ( 'NONE',  ( -8.350000000000008527, 12.50000000000000000, 5.802370205355744659 ) ) ;
#119282=DIRECTION ( 'NONE',  ( 0.000000000000000000, 0.000000000000000000, 1.000000000000000000 ) ) ;
#119283=VERTEX_POINT ( 'NONE', #18470 ) ;
#119284=DIRECTION ( 'NONE',  ( -4.274815082592931898E-19, -0.9999939076577903929, -0.003490651415223739937 ) ) ;
#119286=CIRCLE ( 'NONE', #106762, 0.1000000000000002554 ) ;
#119287=CARTESIAN_POINT ( 'NONE',  ( 9.599999999999914380, 2.500000000000000000, -5.122947341949753763 ) ) ;
#119290=DIRECTION ( 'NONE',  ( 0.000000000000000000, -0.9999939076577903929, 0.003490651415223739937 ) ) ;
#119291=CARTESIAN_POINT ( 'NONE',  ( 3.949999999999942446, 12.50000000000000000, -6.776507416713040577 ) ) ;
#119292=ORIENTED_EDGE ( 'NONE', *, *, #43227, .F. ) ;
#119293=EDGE_LOOP ( 'NONE', ( #47455, #58880, #20940, #108897 ) ) ;
#119294=EDGE_LOOP ( 'NONE', ( #80706, #51937, #93930, #82257 ) ) ;
#119295=ORIENTED_EDGE ( 'NONE', *, *, #56164, .T. ) ;
#119296=CIRCLE ( 'NONE', #21010, 0.1000000000000002554 ) ;
#119297=FACE_OUTER_BOUND ( 'NONE', #99789, .T. ) ;
#119298=CARTESIAN_POINT ( 'NONE',  ( -8.100000000000013856, 12.50000000000000000, -3.983716857408426293 ) ) ;
#119299=CARTESIAN_POINT ( 'NONE',  ( 0.3999999999999619971, 12.50000000000000000, -0.06509327318403752838 ) ) ;
#119300=ORIENTED_EDGE ( 'NONE', *, *, #123411, .F. ) ;
#119301=FACE_BOUND ( 'NONE', #28696, .T. ) ;
#119302=EDGE_LOOP ( 'NONE', ( #108076, #99994 ) ) ;
#119303=FACE_OUTER_BOUND ( 'NONE', #74278, .T. ) ;
#119304=CARTESIAN_POINT ( 'NONE',  ( 0.6499999999999566125, 12.50000000000000000, -6.213873640053564351 ) ) ;
#119305=DIRECTION ( 'NONE',  ( -4.274815082592931898E-19, -0.9999939076577903929, -0.003490651415223739937 ) ) ;
#119306=LINE ( 'NONE', #48015, #74336 ) ;
#119307=CARTESIAN_POINT ( 'NONE',  ( -7.500000000000016875, 2.500000000000000000, 0.5928203230275495006 ) ) ;
#119308=CARTESIAN_POINT ( 'NONE',  ( -8.100000000000013856, 2.500000000000000000, -3.983716857408426293 ) ) ;
#119309=CARTESIAN_POINT ( 'NONE',  ( 6.049999999999934097, 2.500000000000000000, 6.248780366869521430 ) ) ;
#119310=CARTESIAN_POINT ( 'NONE',  ( 6.649999999999929301, 12.50000000000000000, -2.099970236277064473 ) ) ;
#119311=DIRECTION ( 'NONE',  ( 0.000000000000000000, 0.000000000000000000, 1.000000000000000000 ) ) ;
#119312=DIRECTION ( 'NONE',  ( -0.000000000000000000, 1.000000000000000000, -0.000000000000000000 ) ) ;
#119313=VERTEX_POINT ( 'NONE', #8629 ) ;
#119314=ORIENTED_EDGE ( 'NONE', *, *, #3678, .T. ) ;
#119315=ORIENTED_EDGE ( 'NONE', *, *, #5932, .F. ) ;
#119316=ORIENTED_EDGE ( 'NONE', *, *, #121702, .F. ) ;
#119317=CARTESIAN_POINT ( 'NONE',  ( 12.49999999999990585, 2.500000000000000000, 3.537306695894645081 ) ) ;
#119318=AXIS2_PLACEMENT_3D ( 'NONE', #89743, #49836, #91031 ) ;
#119319=EDGE_CURVE ( 'NONE', #66544, #76524, #16306, .T. ) ;
#119320=DIRECTION ( 'NONE',  ( 0.000000000000000000, -0.9999939076577903929, 0.003490651415223739937 ) ) ;
#119321=TOROIDAL_SURFACE ( 'NONE', #98387, 9.000000000000001776, 1.000000000000000000 ) ;
#119322=EDGE_CURVE ( 'NONE', #32088, #124819, #91724, .T. ) ;
#119323=AXIS2_PLACEMENT_3D ( 'NONE', #116130, #103747, #34377 ) ;
#119325=EDGE_LOOP ( 'NONE', ( #42892, #73925, #9753, #42376 ) ) ;
#119326=ORIENTED_EDGE ( 'NONE', *, *, #14691, .T. ) ;
#119327=EDGE_CURVE ( 'NONE', #123047, #118212, #83154, .T. ) ;
#119328=DIRECTION ( 'NONE',  ( -4.274815082592931898E-19, -0.9999939076577903929, -0.003490651415223739937 ) ) ;
#119329=EDGE_CURVE ( 'NONE', #93441, #47940, #32187, .T. ) ;
#119330=CIRCLE ( 'NONE', #16887, 0.06509327318403745899 ) ;
#119331=FACE_OUTER_BOUND ( 'NONE', #28356, .T. ) ;
#119332=LINE ( 'NONE', #89236, #122976 ) ;
#119333=CARTESIAN_POINT ( 'NONE',  ( 7.049999999999928768, 12.50000000000000000, -2.165063509461101710 ) ) ;
#119334=EDGE_CURVE ( 'NONE', #52069, #94129, #43449, .T. ) ;
#119335=PLANE ( 'NONE',  #9545 ) ;
#119336=LINE ( 'NONE', #9398, #10018 ) ;
#119337=AXIS2_PLACEMENT_3D ( 'NONE', #3598, #101809, #23227 ) ;
#119338=PLANE ( 'NONE',  #84491 ) ;
#119339=VERTEX_POINT ( 'NONE', #32824 ) ;
#119340=DIRECTION ( 'NONE',  ( 0.000000000000000000, 0.000000000000000000, 1.000000000000000000 ) ) ;
#119341=ADVANCED_FACE ( 'NONE', ( #52439 ), #110708, .T. ) ;
#119342=ORIENTED_EDGE ( 'NONE', *, *, #38696, .T. ) ;
#119343=EDGE_CURVE ( 'NONE', #37520, #18828, #31518, .T. ) ;
#119344=EDGE_LOOP ( 'NONE', ( #6136, #8395, #99458, #26116 ) ) ;
#119345=VERTEX_POINT ( 'NONE', #42652 ) ;
#119346=LINE ( 'NONE', #29688, #40026 ) ;
#119347=ORIENTED_EDGE ( 'NONE', *, *, #47323, .F. ) ;
#119348=VERTEX_POINT ( 'NONE', #112016 ) ;
#119349=CARTESIAN_POINT ( 'NONE',  ( -4.600000000000028066, 2.500000000000000000, -3.637306695894650055 ) ) ;
#119350=AXIS2_PLACEMENT_3D ( 'NONE', #20816, #119011, #88913 ) ;
#119351=LINE ( 'NONE', #19879, #103947 ) ;
#119352=DIRECTION ( 'NONE',  ( 0.000000000000000000, 0.000000000000000000, -1.000000000000000000 ) ) ;
#119353=FACE_OUTER_BOUND ( 'NONE', #94524, .T. ) ;
#119354=DIRECTION ( 'NONE',  ( 0.000000000000000000, 0.000000000000000000, -1.000000000000000000 ) ) ;
#119355=ORIENTED_EDGE ( 'NONE', *, *, #91256, .T. ) ;
#119356=DIRECTION ( 'NONE',  ( -0.000000000000000000, 1.000000000000000000, -0.000000000000000000 ) ) ;
#119357=AXIS2_PLACEMENT_3D ( 'NONE', #7812, #8447, #96189 ) ;
#119358=AXIS2_PLACEMENT_3D ( 'NONE', #30526, #78971, #39710 ) ;
#119359=ORIENTED_EDGE ( 'NONE', *, *, #116901, .T. ) ;
#119360=CARTESIAN_POINT ( 'NONE',  ( -3.300000000000027800, 12.50000000000000000, -4.395220292106239768 ) ) ;
#119361=VERTEX_POINT ( 'NONE', #11220 ) ;
#119362=DIRECTION ( 'NONE',  ( 0.000000000000000000, 0.000000000000000000, -1.000000000000000000 ) ) ;
#119363=DIRECTION ( 'NONE',  ( -0.000000000000000000, 1.000000000000000000, -0.000000000000000000 ) ) ;
#119364=ORIENTED_EDGE ( 'NONE', *, *, #86204, .T. ) ;
#119365=DIRECTION ( 'NONE',  ( -0.000000000000000000, -1.000000000000000000, -0.000000000000000000 ) ) ;
#119366=FACE_OUTER_BOUND ( 'NONE', #94846, .T. ) ;
#119367=ORIENTED_EDGE ( 'NONE', *, *, #23125, .F. ) ;
#119368=VECTOR ( 'NONE', #68163, 1000.000000000000000 ) ;
#119369=DIRECTION ( 'NONE',  ( -0.000000000000000000, 1.000000000000000000, -0.000000000000000000 ) ) ;
#119370=ORIENTED_EDGE ( 'NONE', *, *, #32070, .T. ) ;
#119372=DIRECTION ( 'NONE',  ( 0.000000000000000000, 0.000000000000000000, -1.000000000000000000 ) ) ;
#119373=CARTESIAN_POINT ( 'NONE',  ( 8.099999999999923261, 2.500000000000000000, 4.083716857408420609 ) ) ;
#119375=DIRECTION ( 'NONE',  ( 0.000000000000000000, 1.000000000000000000, 0.000000000000000000 ) ) ;
#119376=CIRCLE ( 'NONE', #104783, 0.06509327318403745899 ) ;
#119377=AXIS2_PLACEMENT_3D ( 'NONE', #70985, #111548, #92550 ) ;
#119378=DIRECTION ( 'NONE',  ( -0.000000000000000000, -1.000000000000000000, -0.000000000000000000 ) ) ;
#119379=EDGE_CURVE ( 'NONE', #110270, #3522, #20439, .T. ) ;
#119380=VERTEX_POINT ( 'NONE', #40716 ) ;
#119382=ORIENTED_EDGE ( 'NONE', *, *, #113728, .T. ) ;
#119383=DIRECTION ( 'NONE',  ( 0.000000000000000000, 0.000000000000000000, -1.000000000000000000 ) ) ;
#119384=DIRECTION ( 'NONE',  ( -0.000000000000000000, 1.000000000000000000, -0.000000000000000000 ) ) ;
#119385=AXIS2_PLACEMENT_3D ( 'NONE', #62487, #102401, #12702 ) ;
#119386=AXIS2_PLACEMENT_3D ( 'NONE', #116928, #17435, #56709 ) ;
#119387=FACE_OUTER_BOUND ( 'NONE', #104255, .T. ) ;
#119388=CARTESIAN_POINT ( 'NONE',  ( 5.849999999999933920, 12.50000000000000000, -2.165063509461101710 ) ) ;
#119389=FACE_OUTER_BOUND ( 'NONE', #93132, .T. ) ;
#119390=CARTESIAN_POINT ( 'NONE',  ( 5.199999999999937117, 2.500000000000000000, -4.676537180435978769 ) ) ;
#119392=ORIENTED_EDGE ( 'NONE', *, *, #34492, .F. ) ;
#119393=DIRECTION ( 'NONE',  ( 0.000000000000000000, 0.000000000000000000, 1.000000000000000000 ) ) ;
#119394=CARTESIAN_POINT ( 'NONE',  ( -7.950000000000009059, 2.500000000000000000, 6.495190528383297135 ) ) ;
#119395=CARTESIAN_POINT ( 'NONE',  ( -14.79999999999998472, 2.500000000000000000, 0.3464101615137758494 ) ) ;
#119396=EDGE_LOOP ( 'NONE', ( #17898, #117979, #90401, #23923 ) ) ;
#119397=CARTESIAN_POINT ( 'NONE',  ( -3.300000000000027800, 2.500000000000000000, -4.430127018922202176 ) ) ;
#119399=EDGE_LOOP ( 'NONE', ( #28038, #37432, #47792, #31448 ) ) ;
#119400=LINE ( 'NONE', #70326, #126230 ) ;
#119401=AXIS2_PLACEMENT_3D ( 'NONE', #79932, #103294, #64643 ) ;
#119402=CIRCLE ( 'NONE', #79710, 0.06509327318403745899 ) ;
#119403=EDGE_LOOP ( 'NONE', ( #107211, #22740 ) ) ;
#119404=CARTESIAN_POINT ( 'NONE',  ( -8.100000000000013856, 12.50000000000000000, 0.3464101615137736845 ) ) ;
#119405=DIRECTION ( 'NONE',  ( 0.000000000000000000, 1.000000000000000000, 0.000000000000000000 ) ) ;
#119406=VERTEX_POINT ( 'NONE', #1403 ) ;
#119407=EDGE_CURVE ( 'NONE', #98598, #97339, #106218, .T. ) ;
#119408=VECTOR ( 'NONE', #5893, 1000.000000000000000 ) ;
#119409=CARTESIAN_POINT ( 'NONE',  ( -6.050000000000018474, 2.500000000000000000, 2.511473670974873507 ) ) ;
#119410=CIRCLE ( 'NONE', #115285, 0.1000000000000000472 ) ;
#119411=CARTESIAN_POINT ( 'NONE',  ( 10.84999999999991260, 2.500000000000000000, 5.902370205355745192 ) ) ;
#119412=VERTEX_POINT ( 'NONE', #112657 ) ;
#119413=AXIS2_PLACEMENT_3D ( 'NONE', #108871, #57209, #107602 ) ;
#119414=DIRECTION ( 'NONE',  ( 0.000000000000000000, 0.000000000000000000, -1.000000000000000000 ) ) ;
#119415=EDGE_CURVE ( 'NONE', #54453, #35207, #89488, .T. ) ;
#119416=EDGE_CURVE ( 'NONE', #51297, #32033, #122947, .T. ) ;
#119417=VERTEX_POINT ( 'NONE', #62910 ) ;
#119418=EDGE_LOOP ( 'NONE', ( #128259, #28415 ) ) ;
#119419=ORIENTED_EDGE ( 'NONE', *, *, #33421, .F. ) ;
#119420=CARTESIAN_POINT ( 'NONE',  ( 1.849999999999949685, 2.500000000000000000, 1.818653347947321475 ) ) ;
#119421=DIRECTION ( 'NONE',  ( 0.000000000000000000, 1.000000000000000000, 0.000000000000000000 ) ) ;
#119422=ADVANCED_FACE ( 'NONE', ( #2678 ), #13141, .T. ) ;
#119423=EDGE_CURVE ( 'NONE', #54678, #8118, #53896, .T. ) ;
#119424=DIRECTION ( 'NONE',  ( 0.000000000000000000, 0.000000000000000000, 1.000000000000000000 ) ) ;
#119425=EDGE_CURVE ( 'NONE', #12097, #72485, #93022, .T. ) ;
#119426=FACE_BOUND ( 'NONE', #83738, .T. ) ;
#119427=ORIENTED_EDGE ( 'NONE', *, *, #124164, .F. ) ;
#119428=ADVANCED_FACE ( 'NONE', ( #21706 ), #81094, .T. ) ;
#119429=EDGE_CURVE ( 'NONE', #51134, #83059, #97801, .T. ) ;
#119431=LINE ( 'NONE', #109633, #52341 ) ;
#119432=ORIENTED_EDGE ( 'NONE', *, *, #43362, .T. ) ;
#119433=DIRECTION ( 'NONE',  ( -0.000000000000000000, 1.000000000000000000, -0.000000000000000000 ) ) ;
#119434=FACE_OUTER_BOUND ( 'NONE', #106584, .T. ) ;
#119435=DIRECTION ( 'NONE',  ( 0.000000000000000000, -0.9999939076577903929, 0.003490651415223739937 ) ) ;
#119436=FACE_OUTER_BOUND ( 'NONE', #3947, .T. ) ;
#119437=DIRECTION ( 'NONE',  ( -0.000000000000000000, 1.000000000000000000, -0.000000000000000000 ) ) ;
#119438=ADVANCED_FACE ( 'NONE', ( #71419 ), #51814, .T. ) ;
#119439=DIRECTION ( 'NONE',  ( 0.000000000000000000, 1.000000000000000000, 0.000000000000000000 ) ) ;
#119440=DIRECTION ( 'NONE',  ( 0.000000000000000000, 0.000000000000000000, -1.000000000000000000 ) ) ;
#119441=CIRCLE ( 'NONE', #117368, 0.06509327318403745899 ) ;
#119442=CIRCLE ( 'NONE', #102710, 0.06509327318403745899 ) ;
#119443=EDGE_LOOP ( 'NONE', ( #109989, #119650, #65295, #13691 ) ) ;
#119444=EDGE_LOOP ( 'NONE', ( #110409, #44481, #24594, #59818 ) ) ;
#119445=EDGE_LOOP ( 'NONE', ( #127111, #1878, #73644, #114121 ) ) ;
#119446=ORIENTED_EDGE ( 'NONE', *, *, #3599, .F. ) ;
#119447=ORIENTED_EDGE ( 'NONE', *, *, #71510, .T. ) ;
#119448=FACE_OUTER_BOUND ( 'NONE', #74874, .T. ) ;
#119449=DIRECTION ( 'NONE',  ( 0.000000000000000000, 0.000000000000000000, 1.000000000000000000 ) ) ;
#119450=ORIENTED_EDGE ( 'NONE', *, *, #30492, .T. ) ;
#119451=FACE_BOUND ( 'NONE', #30712, .T. ) ;
#119452=CONICAL_SURFACE ( 'NONE', #23305, 0.1000000000000002554, 0.003490658503988666988 ) ;
#119453=CARTESIAN_POINT ( 'NONE',  ( -12.29999999999999716, 2.500000000000000000, -3.983716857408423628 ) ) ;
#119454=CONICAL_SURFACE ( 'NONE', #65068, 0.1000000000000000472, 0.003490658503988666988 ) ;
#119455=VECTOR ( 'NONE', #58703, 1000.000000000000000 ) ;
#119457=DIRECTION ( 'NONE',  ( 0.000000000000000000, 0.000000000000000000, -1.000000000000000000 ) ) ;
#119458=CARTESIAN_POINT ( 'NONE',  ( -2.900000000000030109, 2.500000000000000000, -3.637306695894650055 ) ) ;
#119459=PLANE ( 'NONE',  #74225 ) ;
#119460=FACE_OUTER_BOUND ( 'NONE', #63143, .T. ) ;
#119461=VERTEX_POINT ( 'NONE', #3344 ) ;
#119462=CIRCLE ( 'NONE', #106941, 0.1000000000000002554 ) ;
#119463=VERTEX_POINT ( 'NONE', #14431 ) ;
#119464=CIRCLE ( 'NONE', #8737, 0.06509327318403745899 ) ;
#119466=EDGE_LOOP ( 'NONE', ( #64071, #52936 ) ) ;
#119467=VERTEX_POINT ( 'NONE', #3977 ) ;
#119468=AXIS2_PLACEMENT_3D ( 'NONE', #87510, #117597, #97984 ) ;
#119469=EDGE_CURVE ( 'NONE', #73868, #67061, #43540, .T. ) ;
#119470=CARTESIAN_POINT ( 'NONE',  ( -12.89999999999999147, 2.500000000000000000, -4.430127018922199511 ) ) ;
#119471=CARTESIAN_POINT ( 'NONE',  ( 10.84999999999990905, 2.500000000000000000, -6.395190528383301931 ) ) ;
#119472=ADVANCED_FACE ( 'NONE', ( #106054 ), #18473, .T. ) ;
#119473=ORIENTED_EDGE ( 'NONE', *, *, #84386, .F. ) ;
#119474=CARTESIAN_POINT ( 'NONE',  ( -6.700000000000019718, 2.500000000000000000, 0.09999999999999761857 ) ) ;
#119475=AXIS2_PLACEMENT_3D ( 'NONE', #111551, #31085, #90616 ) ;
#119476=EDGE_CURVE ( 'NONE', #83800, #129352, #5261, .T. ) ;
#119477=DIRECTION ( 'NONE',  ( 0.000000000000000000, 1.000000000000000000, 0.000000000000000000 ) ) ;
#119478=EDGE_CURVE ( 'NONE', #54197, #109690, #104742, .T. ) ;
#119479=CARTESIAN_POINT ( 'NONE',  ( -8.750000000000007105, 12.50000000000000000, 7.188010851410848723 ) ) ;
#119480=CIRCLE ( 'NONE', #88065, 0.06509327318403745899 ) ;
#119481=ADVANCED_BREP_SHAPE_REPRESENTATION ( '', ( #58374, #108296 ), #79070 ) ;
#119483=CARTESIAN_POINT ( 'NONE',  ( 5.649999999999932854, 2.500000000000000000, 1.818653347947321475 ) ) ;
#119484=CARTESIAN_POINT ( 'NONE',  ( 13.14999999999989733, 12.50000000000000000, -1.753560074763288457 ) ) ;
#119486=EDGE_CURVE ( 'NONE', #56423, #61621, #8001, .T. ) ;
#119487=VERTEX_POINT ( 'NONE', #26208 ) ;
#119488=DIRECTION ( 'NONE',  ( 0.000000000000000000, 0.000000000000000000, -1.000000000000000000 ) ) ;
#119489=EDGE_CURVE ( 'NONE', #64836, #28738, #91633, .T. ) ;
#119490=EDGE_CURVE ( 'NONE', #54227, #30984, #34758, .T. ) ;
#119491=ORIENTED_EDGE ( 'NONE', *, *, #3762, .T. ) ;
#119492=EDGE_CURVE ( 'NONE', #23452, #99397, #15057, .T. ) ;
#119493=VERTEX_POINT ( 'NONE', #53731 ) ;
#119494=CARTESIAN_POINT ( 'NONE',  ( -13.29999999999999005, 2.500000000000000000, -4.430127018922199511 ) ) ;
#119495=FACE_OUTER_BOUND ( 'NONE', #80855, .T. ) ;
#119496=DIRECTION ( 'NONE',  ( 0.000000000000000000, 0.000000000000000000, -1.000000000000000000 ) ) ;
#119497=VERTEX_POINT ( 'NONE', #43929 ) ;
#119498=EDGE_CURVE ( 'NONE', #122996, #2794, #103480, .T. ) ;
#119499=VERTEX_POINT ( 'NONE', #16356 ) ;
#119500=DIRECTION ( 'NONE',  ( -0.000000000000000000, 1.000000000000000000, -0.000000000000000000 ) ) ;
#119501=DIRECTION ( 'NONE',  ( -0.000000000000000000, -1.000000000000000000, -0.000000000000000000 ) ) ;
#119502=LINE ( 'NONE', #30515, #8035 ) ;
#119503=CONICAL_SURFACE ( 'NONE', #63076, 0.1000000000000000472, 0.003490658503988666988 ) ;
#119504=DIRECTION ( 'NONE',  ( 0.000000000000000000, 0.000000000000000000, 1.000000000000000000 ) ) ;
#119505=ORIENTED_EDGE ( 'NONE', *, *, #33618, .F. ) ;
#119506=CIRCLE ( 'NONE', #25403, 0.06509327318403741736 ) ;
#119507=CIRCLE ( 'NONE', #46345, 0.09999999999999982514 ) ;
#119508=DIRECTION ( 'NONE',  ( -0.000000000000000000, 1.000000000000000000, -0.000000000000000000 ) ) ;
#119509=EDGE_LOOP ( 'NONE', ( #13467, #80101 ) ) ;
#119510=DIRECTION ( 'NONE',  ( -0.000000000000000000, 1.000000000000000000, -0.000000000000000000 ) ) ;
#119511=CIRCLE ( 'NONE', #35896, 0.1000000000000002554 ) ;
#119512=ORIENTED_EDGE ( 'NONE', *, *, #114447, .T. ) ;
#119513=DIRECTION ( 'NONE',  ( -0.000000000000000000, 1.000000000000000000, -0.000000000000000000 ) ) ;
#119514=VECTOR ( 'NONE', #22611, 1000.000000000000000 ) ;
#119515=DIRECTION ( 'NONE',  ( 0.000000000000000000, 1.000000000000000000, 0.000000000000000000 ) ) ;
#119516=CARTESIAN_POINT ( 'NONE',  ( 10.64999999999990976, 2.500000000000000000, 2.511473670974873507 ) ) ;
#119517=CIRCLE ( 'NONE', #81855, 0.1000000000000000472 ) ;
#119518=ADVANCED_FACE ( 'NONE', ( #44560 ), #93690, .T. ) ;
#119519=DIRECTION ( 'NONE',  ( 0.000000000000000000, 0.000000000000000000, 1.000000000000000000 ) ) ;
#119520=ORIENTED_EDGE ( 'NONE', *, *, #48435, .T. ) ;
#119521=VECTOR ( 'NONE', #58624, 1000.000000000000000 ) ;
#119522=DIRECTION ( 'NONE',  ( 0.000000000000000000, 0.000000000000000000, 1.000000000000000000 ) ) ;
#119523=VERTEX_POINT ( 'NONE', #55660 ) ;
#119524=EDGE_LOOP ( 'NONE', ( #67348, #78199 ) ) ;
#119525=DIRECTION ( 'NONE',  ( -0.000000000000000000, -1.000000000000000000, -0.000000000000000000 ) ) ;
#119526=CARTESIAN_POINT ( 'NONE',  ( 1.849999999999950573, 2.500000000000000000, 2.611473670974873151 ) ) ;
#119527=FACE_OUTER_BOUND ( 'NONE', #96045, .T. ) ;
#119529=CARTESIAN_POINT ( 'NONE',  ( 8.549999999999922551, 2.500000000000000000, 2.511473670974873507 ) ) ;
#119530=DIRECTION ( 'NONE',  ( 0.000000000000000000, 0.000000000000000000, 1.000000000000000000 ) ) ;
#119531=DIRECTION ( 'NONE',  ( 0.000000000000000000, 0.000000000000000000, -1.000000000000000000 ) ) ;
#119532=ADVANCED_FACE ( 'NONE', ( #123738 ), #112576, .T. ) ;
#119533=CARTESIAN_POINT ( 'NONE',  ( 10.84999999999991260, 12.50000000000000000, 5.737276932171707422 ) ) ;
#119534=CARTESIAN_POINT ( 'NONE',  ( 6.449999999999931788, 12.50000000000000000, -6.083687093685488989 ) ) ;
#119535=CIRCLE ( 'NONE', #65243, 0.1000000000000002554 ) ;
#119536=CONICAL_SURFACE ( 'NONE', #67274, 0.09999999999999982514, 0.003490658503988666988 ) ;
#119537=ORIENTED_EDGE ( 'NONE', *, *, #107997, .T. ) ;
#119538=DIRECTION ( 'NONE',  ( 0.000000000000000000, 0.000000000000000000, 1.000000000000000000 ) ) ;
#119539=EDGE_CURVE ( 'NONE', #89688, #32515, #37275, .T. ) ;
#119540=CARTESIAN_POINT ( 'NONE',  ( -10.45000000000000107, 2.500000000000000000, 2.165063509461097713 ) ) ;
#119541=CARTESIAN_POINT ( 'NONE',  ( 9.599999999999917932, 2.500000000000000000, -2.276824562219559311E-15 ) ) ;
#119542=DIRECTION ( 'NONE',  ( 0.000000000000000000, 0.000000000000000000, 1.000000000000000000 ) ) ;
#119543=DIRECTION ( 'NONE',  ( 0.000000000000000000, -0.9999939076577903929, 0.003490651415223739937 ) ) ;
#119544=VECTOR ( 'NONE', #83689, 1000.000000000000000 ) ;
#119545=ORIENTED_EDGE ( 'NONE', *, *, #64008, .F. ) ;
#119546=DIRECTION ( 'NONE',  ( 0.000000000000000000, 0.000000000000000000, -1.000000000000000000 ) ) ;
#119547=AXIS2_PLACEMENT_3D ( 'NONE', #26343, #44692, #85877 ) ;
#119548=AXIS2_PLACEMENT_3D ( 'NONE', #72398, #93319, #92670 ) ;
#119549=CARTESIAN_POINT ( 'NONE',  ( 0.4499999999999573785, 12.50000000000000000, -6.495190528383302464 ) ) ;
#119550=LINE ( 'NONE', #127457, #334 ) ;
#119551=ORIENTED_EDGE ( 'NONE', *, *, #41172, .F. ) ;
#119552=AXIS2_PLACEMENT_3D ( 'NONE', #24601, #4282, #64513 ) ;
#119556=VERTEX_POINT ( 'NONE', #35387 ) ;
#119557=CONICAL_SURFACE ( 'NONE', #84062, 0.09999999999999999167, 0.003490658503988666988 ) ;
#119558=VERTEX_POINT ( 'NONE', #25538 ) ;
#119559=VECTOR ( 'NONE', #57342, 1000.000000000000000 ) ;
#119560=DIRECTION ( 'NONE',  ( 0.000000000000000000, 0.000000000000000000, 1.000000000000000000 ) ) ;
#119561=CIRCLE ( 'NONE', #111236, 0.1000000000000002554 ) ;
#119562=CARTESIAN_POINT ( 'NONE',  ( 8.099999999999923261, 2.500000000000000000, -4.776537180435978414 ) ) ;
#119563=CARTESIAN_POINT ( 'NONE',  ( -13.74999999999995381, 12.50000000000000000, 2.165063509461101265 ) ) ;
#119564=DIRECTION ( 'NONE',  ( 0.000000000000000000, -0.000000000000000000, 1.000000000000000000 ) ) ;
#119565=ORIENTED_EDGE ( 'NONE', *, *, #80193, .F. ) ;
#119566=EDGE_CURVE ( 'NONE', #83925, #79983, #68651, .T. ) ;
#119567=AXIS2_PLACEMENT_3D ( 'NONE', #112709, #110756, #23036 ) ;
#119568=DIRECTION ( 'NONE',  ( 0.000000000000000000, 0.000000000000000000, 1.000000000000000000 ) ) ;
#119569=ORIENTED_EDGE ( 'NONE', *, *, #41476, .F. ) ;
#119570=DIRECTION ( 'NONE',  ( 0.000000000000000000, 1.000000000000000000, 0.000000000000000000 ) ) ;
#119571=CARTESIAN_POINT ( 'NONE',  ( 19.08853762629104978, 0.5565172523999983856, 4.470057054643344685 ) ) ;
#119572=DIRECTION ( 'NONE',  ( 0.000000000000000000, 0.000000000000000000, 1.000000000000000000 ) ) ;
#119573=CARTESIAN_POINT ( 'NONE',  ( -5.200000000000022382, 2.500000000000000000, 0.3464101615137735735 ) ) ;
#119574=ORIENTED_EDGE ( 'NONE', *, *, #13179, .T. ) ;
#119575=ORIENTED_EDGE ( 'NONE', *, *, #86951, .F. ) ;
#119576=VERTEX_POINT ( 'NONE', #45851 ) ;
#119577=EDGE_LOOP ( 'NONE', ( #124461, #124903, #8688, #27103 ) ) ;
#119578=ORIENTED_EDGE ( 'NONE', *, *, #79504, .F. ) ;
#119579=DIRECTION ( 'NONE',  ( 0.000000000000000000, -0.000000000000000000, 1.000000000000000000 ) ) ;
#119580=LINE ( 'NONE', #19456, #104162 ) ;
#119581=ADVANCED_FACE ( 'NONE', ( #85757 ), #70705, .T. ) ;
#119582=EDGE_CURVE ( 'NONE', #56299, #50883, #121595, .T. ) ;
#119583=DIRECTION ( 'NONE',  ( -0.000000000000000000, -1.000000000000000000, -0.000000000000000000 ) ) ;
#119584=EDGE_CURVE ( 'NONE', #110814, #51534, #85375, .T. ) ;
#119585=FACE_BOUND ( 'NONE', #98401, .T. ) ;
#119586=EDGE_CURVE ( 'NONE', #116584, #70542, #28957, .T. ) ;
#119587=DIRECTION ( 'NONE',  ( 0.000000000000000000, 0.000000000000000000, 1.000000000000000000 ) ) ;
#119588=CARTESIAN_POINT ( 'NONE',  ( 12.04999999999990834, 2.500000000000000000, -2.165063509461101710 ) ) ;
#119589=DIRECTION ( 'NONE',  ( 0.000000000000000000, -0.000000000000000000, 1.000000000000000000 ) ) ;
#119590=DIRECTION ( 'NONE',  ( 0.000000000000000000, 1.000000000000000000, 0.000000000000000000 ) ) ;
#119591=AXIS2_PLACEMENT_3D ( 'NONE', #109118, #19464, #90786 ) ;
#119592=AXIS2_PLACEMENT_3D ( 'NONE', #49162, #19016, #58964 ) ;
#119593=CARTESIAN_POINT ( 'NONE',  ( -0.6500000000000394351, 12.50000000000000000, 6.841600689897072485 ) ) ;
#119594=LINE ( 'NONE', #88859, #783 ) ;
#119595=ADVANCED_FACE ( 'NONE', ( #33863 ), #108355, .T. ) ;
#119596=DIRECTION ( 'NONE',  ( 0.000000000000000000, 0.000000000000000000, 1.000000000000000000 ) ) ;
#119597=EDGE_CURVE ( 'NONE', #85559, #96252, #102104, .T. ) ;
#119598=VECTOR ( 'NONE', #42833, 1000.000000000000000 ) ;
#119599=ADVANCED_FACE ( 'NONE', ( #43080 ), #123038, .T. ) ;
#119600=AXIS2_PLACEMENT_3D ( 'NONE', #2016, #41962, #62251 ) ;
#119601=CARTESIAN_POINT ( 'NONE',  ( -7.700000000000012612, 12.50000000000000000, 4.676537180435972552 ) ) ;
#119602=VECTOR ( 'NONE', #13723, 1000.000000000000000 ) ;
#119604=EDGE_LOOP ( 'NONE', ( #49738, #73200 ) ) ;
#119605=ORIENTED_EDGE ( 'NONE', *, *, #127322, .T. ) ;
#119606=ORIENTED_EDGE ( 'NONE', *, *, #72377, .T. ) ;
#119607=CIRCLE ( 'NONE', #102873, 0.1000000000000000472 ) ;
#119608=LINE ( 'NONE', #99988, #37644 ) ;
#119609=VECTOR ( 'NONE', #77172, 1000.000000000000000 ) ;
#119610=FACE_OUTER_BOUND ( 'NONE', #79797, .T. ) ;
#119611=FACE_BOUND ( 'NONE', #78693, .T. ) ;
#119612=AXIS2_PLACEMENT_3D ( 'NONE', #54187, #15526, #45013 ) ;
#119613=DIRECTION ( 'NONE',  ( 0.000000000000000000, 0.000000000000000000, 1.000000000000000000 ) ) ;
#119614=ORIENTED_EDGE ( 'NONE', *, *, #31895, .T. ) ;
#119615=CARTESIAN_POINT ( 'NONE',  ( -13.94999999999998685, 2.500000000000000000, -2.411473670974875638 ) ) ;
#119616=DIRECTION ( 'NONE',  ( 0.000000000000000000, 1.000000000000000000, 0.000000000000000000 ) ) ;
#119617=DIRECTION ( 'NONE',  ( -0.000000000000000000, 1.000000000000000000, -0.000000000000000000 ) ) ;
#119618=CARTESIAN_POINT ( 'NONE',  ( 6.449999999999931788, 2.500000000000000000, 6.148780366869520009 ) ) ;
#119619=ORIENTED_EDGE ( 'NONE', *, *, #12192, .T. ) ;
#119620=FACE_OUTER_BOUND ( 'NONE', #103337, .T. ) ;
#119621=ORIENTED_EDGE ( 'NONE', *, *, #3509, .T. ) ;
#119622=ORIENTED_EDGE ( 'NONE', *, *, #108875, .F. ) ;
#119623=CARTESIAN_POINT ( 'NONE',  ( 1.249999999999950262, 2.500000000000000000, 7.088010851410848190 ) ) ;
#119624=FACE_OUTER_BOUND ( 'NONE', #82823, .T. ) ;
#119625=ORIENTED_EDGE ( 'NONE', *, *, #59498, .F. ) ;
#119626=AXIS2_PLACEMENT_3D ( 'NONE', #80127, #68360, #18622 ) ;
#119627=CARTESIAN_POINT ( 'NONE',  ( -10.40000000000000213, 12.50000000000000000, 0.6277270498435120194 ) ) ;
#119628=CARTESIAN_POINT ( 'NONE',  ( -7.100000000000017408, 2.500000000000000000, -5.022947341949754119 ) ) ;
#119629=ORIENTED_EDGE ( 'NONE', *, *, #124723, .T. ) ;
#119630=CARTESIAN_POINT ( 'NONE',  ( -0.4000000000000396572, 2.500000000000000000, 4.330127018922196314 ) ) ;
#119631=VERTEX_POINT ( 'NONE', #120960 ) ;
#119632=FACE_OUTER_BOUND ( 'NONE', #40468, .T. ) ;
#119633=EDGE_CURVE ( 'NONE', #15440, #82143, #24742, .T. ) ;
#119634=ORIENTED_EDGE ( 'NONE', *, *, #109735, .F. ) ;
#119635=CARTESIAN_POINT ( 'NONE',  ( 0.8499999999999557909, 2.500000000000000000, -6.495190528383302464 ) ) ;
#119637=EDGE_CURVE ( 'NONE', #120463, #78289, #92139, .T. ) ;
#119638=AXIS2_PLACEMENT_3D ( 'NONE', #70870, #70227, #110779 ) ;
#119639=EDGE_LOOP ( 'NONE', ( #48242, #59720, #74820, #117331 ) ) ;
#119640=CONICAL_SURFACE ( 'NONE', #98806, 0.09999999999999982514, 0.003490658503988666988 ) ;
#119641=DIRECTION ( 'NONE',  ( 0.000000000000000000, 0.000000000000000000, -1.000000000000000000 ) ) ;
#119642=ADVANCED_FACE ( 'NONE', ( #11652 ), #113066, .T. ) ;
#119643=ORIENTED_EDGE ( 'NONE', *, *, #82552, .F. ) ;
#119644=DIRECTION ( 'NONE',  ( 0.000000000000000000, 0.000000000000000000, 1.000000000000000000 ) ) ;
#119645=DIRECTION ( 'NONE',  ( -0.000000000000000000, 1.000000000000000000, -0.000000000000000000 ) ) ;
#119646=DIRECTION ( 'NONE',  ( 0.000000000000000000, 0.000000000000000000, 1.000000000000000000 ) ) ;
#119647=CARTESIAN_POINT ( 'NONE',  ( -6.250000000000015987, 12.50000000000000000, 1.472243186433545459 ) ) ;
#119648=DIRECTION ( 'NONE',  ( 0.000000000000000000, 0.000000000000000000, 1.000000000000000000 ) ) ;
#119649=CIRCLE ( 'NONE', #59031, 0.06509327318403741736 ) ;
#119650=ORIENTED_EDGE ( 'NONE', *, *, #40572, .T. ) ;
#119651=EDGE_CURVE ( 'NONE', #91958, #93869, #99956, .T. ) ;
#119652=ORIENTED_EDGE ( 'NONE', *, *, #78886, .T. ) ;
#119653=AXIS2_PLACEMENT_3D ( 'NONE', #52468, #13173, #75330 ) ;
#119654=EDGE_LOOP ( 'NONE', ( #62264, #2149, #121841, #99206 ) ) ;
#119655=FACE_OUTER_BOUND ( 'NONE', #23182, .T. ) ;
#119656=DIRECTION ( 'NONE',  ( 0.000000000000000000, 1.000000000000000000, 0.000000000000000000 ) ) ;
#119657=VECTOR ( 'NONE', #22302, 1000.000000000000000 ) ;
#119658=CIRCLE ( 'NONE', #127981, 0.09999999999999982514 ) ;
#119659=CARTESIAN_POINT ( 'NONE',  ( 8.549999999999918998, 2.500000000000000000, -1.818653347947326138 ) ) ;
#119660=ORIENTED_EDGE ( 'NONE', *, *, #62147, .T. ) ;
#119661=ORIENTED_EDGE ( 'NONE', *, *, #101620, .T. ) ;
#119662=ORIENTED_EDGE ( 'NONE', *, *, #120180, .T. ) ;
#119663=DIRECTION ( 'NONE',  ( 0.000000000000000000, 1.000000000000000000, 0.000000000000000000 ) ) ;
#119664=CIRCLE ( 'NONE', #107137, 0.06509327318403745899 ) ;
#119665=EDGE_LOOP ( 'NONE', ( #39709, #10893 ) ) ;
#119666=CARTESIAN_POINT ( 'NONE',  ( -1.050000000000037348, 2.500000000000000000, -2.511473670974877948 ) ) ;
#119667=DIRECTION ( 'NONE',  ( 0.000000000000000000, 1.000000000000000000, 0.000000000000000000 ) ) ;
#119668=AXIS2_PLACEMENT_3D ( 'NONE', #49781, #47842, #87095 ) ;
#119669=CARTESIAN_POINT ( 'NONE',  ( 13.94999999999989626, 12.50000000000000000, 2.511473670974873507 ) ) ;
#119670=CARTESIAN_POINT ( 'NONE',  ( -10.45000000000000462, 2.500000000000000000, -6.395190528383298378 ) ) ;
#119671=DIRECTION ( 'NONE',  ( 0.000000000000000000, 0.000000000000000000, 1.000000000000000000 ) ) ;
#119672=CARTESIAN_POINT ( 'NONE',  ( -6.850000000000013856, 2.500000000000000000, 2.511473670974873507 ) ) ;
#119673=DIRECTION ( 'NONE',  ( 0.000000000000000000, 0.000000000000000000, 1.000000000000000000 ) ) ;
#119674=EDGE_LOOP ( 'NONE', ( #100736, #110049, #90427, #77985 ) ) ;
#119675=ORIENTED_EDGE ( 'NONE', *, *, #81486, .T. ) ;
#119676=CARTESIAN_POINT ( 'NONE',  ( -14.14999999999998614, 2.500000000000000000, -2.165063509461099489 ) ) ;
#119677=ORIENTED_EDGE ( 'NONE', *, *, #128961, .F. ) ;
#119678=ORIENTED_EDGE ( 'NONE', *, *, #62292, .T. ) ;
#119679=AXIS2_PLACEMENT_3D ( 'NONE', #94417, #114706, #25047 ) ;
#119682=DIRECTION ( 'NONE',  ( 0.000000000000000000, 1.000000000000000000, 0.000000000000000000 ) ) ;
#119683=DIRECTION ( 'NONE',  ( 0.000000000000000000, 0.000000000000000000, 1.000000000000000000 ) ) ;
#119684=CARTESIAN_POINT ( 'NONE',  ( 3.149999999999946176, 12.50000000000000000, -6.148780366869526226 ) ) ;
#119685=ADVANCED_FACE ( 'NONE', ( #31953 ), #111116, .T. ) ;
#119686=CONICAL_SURFACE ( 'NONE', #128108, 0.1000000000000002554, 0.003490658503988666988 ) ;
#119687=CARTESIAN_POINT ( 'NONE',  ( 4.149999999999938183, 2.500000000000000000, 2.265063509461097357 ) ) ;
#119688=CARTESIAN_POINT ( 'NONE',  ( 8.149999999999923972, 12.50000000000000000, -6.148780366869526226 ) ) ;
#119689=AXIS2_PLACEMENT_3D ( 'NONE', #22277, #34011, #91638 ) ;
#119690=AXIS2_PLACEMENT_3D ( 'NONE', #85078, #15017, #115152 ) ;
#119691=DIRECTION ( 'NONE',  ( -0.000000000000000000, -1.000000000000000000, -0.000000000000000000 ) ) ;
#119692=AXIS2_PLACEMENT_3D ( 'NONE', #23576, #6474, #34050 ) ;
#119693=ORIENTED_EDGE ( 'NONE', *, *, #71457, .F. ) ;
#119694=AXIS2_PLACEMENT_3D ( 'NONE', #54204, #11690, #23444 ) ;
#119695=AXIS2_PLACEMENT_3D ( 'NONE', #63853, #103778, #101203 ) ;
#119696=VERTEX_POINT ( 'NONE', #112446 ) ;
#119697=CIRCLE ( 'NONE', #73722, 0.1000000000000002554 ) ;
#119698=ADVANCED_FACE ( 'NONE', ( #61419 ), #49890, .T. ) ;
#119699=CIRCLE ( 'NONE', #73725, 0.1000000000000002554 ) ;
#119700=VERTEX_POINT ( 'NONE', #91503 ) ;
#119701=ADVANCED_FACE ( 'NONE', ( #22785 ), #71878, .T. ) ;
#119702=ORIENTED_EDGE ( 'NONE', *, *, #26984, .T. ) ;
#119703=DIRECTION ( 'NONE',  ( 0.000000000000000000, 1.000000000000000000, 0.000000000000000000 ) ) ;
#119704=LINE ( 'NONE', #58234, #81279 ) ;
#119705=AXIS2_PLACEMENT_3D ( 'NONE', #51464, #42279, #22649 ) ;
#119706=ORIENTED_EDGE ( 'NONE', *, *, #93035, .F. ) ;
#119707=CARTESIAN_POINT ( 'NONE',  ( -11.44999999999999751, 2.500000000000000000, 6.741600689897071952 ) ) ;
#119708=CARTESIAN_POINT ( 'NONE',  ( -4.999999999999986677, 12.50000000000000000, 4.330127018922196314 ) ) ;
#119709=DIRECTION ( 'NONE',  ( -4.274815082592931898E-19, -0.9999939076577903929, -0.003490651415223739937 ) ) ;
#119710=CARTESIAN_POINT ( 'NONE',  ( -4.400000000000025224, 2.500000000000000000, -0.3464101615137783474 ) ) ;
#119711=ORIENTED_EDGE ( 'NONE', *, *, #84438, .F. ) ;
#119712=ADVANCED_FACE ( 'NONE', ( #63334 ), #53987, .T. ) ;
#119713=CARTESIAN_POINT ( 'NONE',  ( -3.150000000000029665, 2.500000000000000000, 6.941600689897073018 ) ) ;
#119714=CONICAL_SURFACE ( 'NONE', #4773, 0.1000000000000000472, 0.003490658503988666988 ) ;
#119716=EDGE_LOOP ( 'NONE', ( #26523, #17020 ) ) ;
#119717=EDGE_LOOP ( 'NONE', ( #66957, #20576, #111075, #23872 ) ) ;
#119718=EDGE_LOOP ( 'NONE', ( #20522, #77836 ) ) ;
#119719=VERTEX_POINT ( 'NONE', #12283 ) ;
#119720=CARTESIAN_POINT ( 'NONE',  ( 16.56576425165006583, -1.500000000000000666, 6.084390597445813675 ) ) ;
#119721=CARTESIAN_POINT ( 'NONE',  ( 4.799999999999935874, 2.500000000000000000, 0.4464101615137735513 ) ) ;
#119722=CIRCLE ( 'NONE', #111393, 0.06509327318403745899 ) ;
#119723=CARTESIAN_POINT ( 'NONE',  ( -3.150000000000032330, 2.500000000000000000, -6.148780366869526226 ) ) ;
#119724=AXIS2_PLACEMENT_3D ( 'NONE', #112068, #23681, #43337 ) ;
#119725=ADVANCED_FACE ( 'NONE', ( #42418 ), #104154, .T. ) ;
#119726=VERTEX_POINT ( 'NONE', #43717 ) ;
#119727=DIRECTION ( 'NONE',  ( 0.000000000000000000, 0.000000000000000000, 1.000000000000000000 ) ) ;
#119728=CARTESIAN_POINT ( 'NONE',  ( 3.349999999999941913, 2.500000000000000000, 6.395190528383296602 ) ) ;
#119729=PLANE ( 'NONE',  #127829 ) ;
#119730=PLANE ( 'NONE',  #67195 ) ;
#119731=AXIS2_PLACEMENT_3D ( 'NONE', #20270, #79208, #60223 ) ;
#119732=VECTOR ( 'NONE', #108578, 1000.000000000000000 ) ;
#119733=VECTOR ( 'NONE', #77945, 1000.000000000000000 ) ;
#119734=ADVANCED_FACE ( 'NONE', ( #6314 ), #120874, .T. ) ;
#119735=ORIENTED_EDGE ( 'NONE', *, *, #97767, .F. ) ;
#119736=LINE ( 'NONE', #73064, #112704 ) ;
#119737=CIRCLE ( 'NONE', #100958, 0.09999999999999982514 ) ;
#119738=ORIENTED_EDGE ( 'NONE', *, *, #18192, .T. ) ;
#119739=ORIENTED_EDGE ( 'NONE', *, *, #17297, .T. ) ;
#119740=DIRECTION ( 'NONE',  ( -0.000000000000000000, 1.000000000000000000, -0.000000000000000000 ) ) ;
#119741=EDGE_CURVE ( 'NONE', #112974, #20780, #64441, .T. ) ;
#119742=EDGE_CURVE ( 'NONE', #128672, #101827, #74918, .T. ) ;
#119743=CARTESIAN_POINT ( 'NONE',  ( -2.100000000000033396, 2.500000000000000000, -0.6928203230275542523 ) ) ;
#119744=EDGE_CURVE ( 'NONE', #75000, #124476, #86165, .T. ) ;
#119745=FACE_BOUND ( 'NONE', #34269, .T. ) ;
#119746=ADVANCED_FACE ( 'NONE', ( #116282 ), #49992, .T. ) ;
#119747=LINE ( 'NONE', #30754, #17884 ) ;
#119748=AXIS2_PLACEMENT_3D ( 'NONE', #4458, #71285, #32043 ) ;
#119749=DIRECTION ( 'NONE',  ( 0.000000000000000000, 1.000000000000000000, 0.000000000000000000 ) ) ;
#119750=CONICAL_SURFACE ( 'NONE', #19394, 0.1000000000000002554, 0.003490658503988666988 ) ;
#119751=DIRECTION ( 'NONE',  ( -0.000000000000000000, -1.000000000000000000, -0.000000000000000000 ) ) ;
#119752=CIRCLE ( 'NONE', #33991, 0.1000000000000002554 ) ;
#119753=ADVANCED_FACE ( 'NONE', ( #24702 ), #4378, .T. ) ;
#119754=CARTESIAN_POINT ( 'NONE',  ( 0.6499999999999561684, 12.50000000000000000, 1.883746621131358934 ) ) ;
#119755=DIRECTION ( 'NONE',  ( 0.000000000000000000, 0.000000000000000000, 1.000000000000000000 ) ) ;
#119756=EDGE_CURVE ( 'NONE', #29817, #62380, #41581, .T. ) ;
#119757=DIRECTION ( 'NONE',  ( 0.000000000000000000, 1.000000000000000000, 0.000000000000000000 ) ) ;
#119758=AXIS2_PLACEMENT_3D ( 'NONE', #103198, #13517, #53469 ) ;
#119759=CARTESIAN_POINT ( 'NONE',  ( 4.399999999999939071, 2.500000000000000000, -0.2464101615137782308 ) ) ;
#119760=VERTEX_POINT ( 'NONE', #115639 ) ;
#119761=CARTESIAN_POINT ( 'NONE',  ( -1.450000000000035927, 2.500000000000000000, -6.148780366869526226 ) ) ;
#119762=EDGE_CURVE ( 'NONE', #43692, #129541, #64528, .T. ) ;
#119763=ADVANCED_FACE ( 'NONE', ( #77016 ), #31112, .T. ) ;
#119764=FACE_OUTER_BOUND ( 'NONE', #68984, .T. ) ;
#119765=AXIS2_PLACEMENT_3D ( 'NONE', #121555, #31908, #92099 ) ;
#119766=VERTEX_POINT ( 'NONE', #34541 ) ;
#119767=ORIENTED_EDGE ( 'NONE', *, *, #105442, .T. ) ;
#119768=DIRECTION ( 'NONE',  ( -0.000000000000000000, -1.000000000000000000, -0.000000000000000000 ) ) ;
#119769=EDGE_CURVE ( 'NONE', #74448, #44266, #52032, .T. ) ;
#119770=CARTESIAN_POINT ( 'NONE',  ( 10.59999999999990905, 12.50000000000000000, 3.918623584224382839 ) ) ;
#119771=FACE_BOUND ( 'NONE', #123071, .T. ) ;
#119772=EDGE_CURVE ( 'NONE', #103467, #39602, #60356, .T. ) ;
#119773=DIRECTION ( 'NONE',  ( -0.000000000000000000, 1.000000000000000000, -0.000000000000000000 ) ) ;
#119774=DIRECTION ( 'NONE',  ( 0.000000000000000000, -0.000000000000000000, 1.000000000000000000 ) ) ;
#119775=CONICAL_SURFACE ( 'NONE', #88361, 0.1000000000000000472, 0.003490658503988666988 ) ;
#119776=VERTEX_POINT ( 'NONE', #116923 ) ;
#119777=DIRECTION ( 'NONE',  ( 0.000000000000000000, 0.000000000000000000, 1.000000000000000000 ) ) ;
#119778=CIRCLE ( 'NONE', #40378, 0.09999999999999982514 ) ;
#119779=CARTESIAN_POINT ( 'NONE',  ( 4.999999999999936939, 2.500000000000000000, -3.637306695894650055 ) ) ;
#119780=ORIENTED_EDGE ( 'NONE', *, *, #103535, .F. ) ;
#119782=CARTESIAN_POINT ( 'NONE',  ( -7.300000000000014921, 2.500000000000000000, 4.676537180435972552 ) ) ;
#119783=AXIS2_PLACEMENT_3D ( 'NONE', #71113, #120860, #29911 ) ;
#119784=AXIS2_PLACEMENT_3D ( 'NONE', #65389, #47062, #96144 ) ;
#119785=CIRCLE ( 'NONE', #48699, 0.1000000000000000472 ) ;
#119787=DIRECTION ( 'NONE',  ( 0.000000000000000000, 1.000000000000000000, 0.000000000000000000 ) ) ;
#119788=AXIS2_PLACEMENT_3D ( 'NONE', #87187, #48576, #101 ) ;
#119789=AXIS2_PLACEMENT_3D ( 'NONE', #100558, #112324, #62588 ) ;
#119790=ORIENTED_EDGE ( 'NONE', *, *, #86536, .T. ) ;
#119791=VECTOR ( 'NONE', #92563, 1000.000000000000000 ) ;
#119792=CARTESIAN_POINT ( 'NONE',  ( -5.400000000000019895, 2.500000000000000000, 4.430127018922196847 ) ) ;
#119793=LINE ( 'NONE', #49145, #14277 ) ;
#119794=CARTESIAN_POINT ( 'NONE',  ( 6.249999999999967137, 2.500000000000000000, -2.265063509461101798 ) ) ;
#119795=AXIS2_PLACEMENT_3D ( 'NONE', #92788, #90842, #1171 ) ;
#119796=DIRECTION ( 'NONE',  ( 0.000000000000000000, 0.000000000000000000, -1.000000000000000000 ) ) ;
#119797=AXIS2_PLACEMENT_3D ( 'NONE', #84598, #13907, #55776 ) ;
#119798=ORIENTED_EDGE ( 'NONE', *, *, #113394, .F. ) ;
#119799=ORIENTED_EDGE ( 'NONE', *, *, #14574, .F. ) ;
#119800=CARTESIAN_POINT ( 'NONE',  ( 12.49999999999990585, 12.50000000000000000, 3.637306695894644726 ) ) ;
#119803=DIRECTION ( 'NONE',  ( -0.000000000000000000, 1.000000000000000000, -0.000000000000000000 ) ) ;
#119804=CARTESIAN_POINT ( 'NONE',  ( 87.50000000000001421, -7.032605354647523122, 2.693424153406290600 ) ) ;
#119805=EDGE_CURVE ( 'NONE', #44454, #108519, #56704, .T. ) ;
#119806=LINE ( 'NONE', #38700, #92649 ) ;
#119807=ORIENTED_EDGE ( 'NONE', *, *, #101348, .F. ) ;
#119808=DIRECTION ( 'NONE',  ( -4.274815082592931898E-19, -0.9999939076577903929, -0.003490651415223739937 ) ) ;
#119809=ADVANCED_FACE ( 'NONE', ( #16779 ), #102203, .T. ) ;
#119810=DIRECTION ( 'NONE',  ( 0.000000000000000000, 0.000000000000000000, -1.000000000000000000 ) ) ;
#119811=CARTESIAN_POINT ( 'NONE',  ( 1.249999999999952482, 2.500000000000000000, -5.802370205355749988 ) ) ;
#119812=CARTESIAN_POINT ( 'NONE',  ( -10.20000000000000462, 2.500000000000000000, -4.576537180435972907 ) ) ;
#119813=DIRECTION ( 'NONE',  ( 0.000000000000000000, 1.000000000000000000, 0.000000000000000000 ) ) ;
#119814=CARTESIAN_POINT ( 'NONE',  ( -6.250000000000019540, 12.50000000000000000, -7.188010851410854052 ) ) ;
#119815=AXIS2_PLACEMENT_3D ( 'NONE', #71441, #59731, #122 ) ;
#119816=ORIENTED_EDGE ( 'NONE', *, *, #73, .F. ) ;
#119817=EDGE_LOOP ( 'NONE', ( #43061, #125838 ) ) ;
#119818=DIRECTION ( 'NONE',  ( 0.000000000000000000, 1.000000000000000000, 0.000000000000000000 ) ) ;
#119819=VERTEX_POINT ( 'NONE', #54786 ) ;
#119820=CARTESIAN_POINT ( 'NONE',  ( 17.50000000000000000, 2.500000000000000000, 4.000000000000000888 ) ) ;
#119821=ORIENTED_EDGE ( 'NONE', *, *, #9936, .F. ) ;
#119822=VERTEX_POINT ( 'NONE', #94718 ) ;
#119823=VERTEX_POINT ( 'NONE', #124836 ) ;
#119824=DIRECTION ( 'NONE',  ( -4.274815082592931898E-19, -0.9999939076577903929, -0.003490651415223739937 ) ) ;
#119825=CONICAL_SURFACE ( 'NONE', #103099, 0.1000000000000002554, 0.003490658503988666988 ) ;
#119826=DIRECTION ( 'NONE',  ( 0.000000000000000000, -0.000000000000000000, 1.000000000000000000 ) ) ;
#119827=CIRCLE ( 'NONE', #63397, 0.09999999999999982514 ) ;
#119828=FACE_OUTER_BOUND ( 'NONE', #17955, .T. ) ;
#119829=FACE_OUTER_BOUND ( 'NONE', #85666, .T. ) ;
#119830=DIRECTION ( 'NONE',  ( -4.274815082592931898E-19, -0.9999939076577903929, -0.003490651415223739937 ) ) ;
#119831=DIRECTION ( 'NONE',  ( -0.000000000000000000, 1.000000000000000000, -0.000000000000000000 ) ) ;
#119832=CARTESIAN_POINT ( 'NONE',  ( -3.350000000000031619, 2.500000000000000000, -5.802370205355749988 ) ) ;
#119833=LINE ( 'NONE', #50447, #84266 ) ;
#119834=VECTOR ( 'NONE', #35894, 1000.000000000000000 ) ;
#119835=AXIS2_PLACEMENT_3D ( 'NONE', #105842, #26641, #35189 ) ;
#119836=CARTESIAN_POINT ( 'NONE',  ( 6.249999999999932498, 2.500000000000000000, -5.902370205355750521 ) ) ;
#119837=ORIENTED_EDGE ( 'NONE', *, *, #95058, .T. ) ;
#119838=VECTOR ( 'NONE', #128708, 1000.000000000000000 ) ;
#119839=ORIENTED_EDGE ( 'NONE', *, *, #93634, .T. ) ;
#119840=AXIS2_PLACEMENT_3D ( 'NONE', #65465, #58721, #105404 ) ;
#119841=DIRECTION ( 'NONE',  ( 0.000000000000000000, 1.000000000000000000, 0.000000000000000000 ) ) ;
#119842=ORIENTED_EDGE ( 'NONE', *, *, #106983, .T. ) ;
#119843=ORIENTED_EDGE ( 'NONE', *, *, #24299, .F. ) ;
#119844=DIRECTION ( 'NONE',  ( 0.000000000000000000, 0.000000000000000000, -1.000000000000000000 ) ) ;
#119845=DIRECTION ( 'NONE',  ( 0.000000000000000000, 0.000000000000000000, 1.000000000000000000 ) ) ;
#119846=EDGE_CURVE ( 'NONE', #34866, #28525, #35180, .T. ) ;
#119848=FACE_OUTER_BOUND ( 'NONE', #107885, .T. ) ;
#119849=CONICAL_SURFACE ( 'NONE', #17423, 0.1000000000000002554, 0.003490658503988666988 ) ;
#119850=DIRECTION ( 'NONE',  ( -0.000000000000000000, -1.000000000000000000, -0.000000000000000000 ) ) ;
#119851=AXIS2_PLACEMENT_3D ( 'NONE', #80103, #38918, #89271 ) ;
#119852=AXIS2_PLACEMENT_3D ( 'NONE', #71857, #101955, #10346 ) ;
#119853=DIRECTION ( 'NONE',  ( 0.000000000000000000, 0.000000000000000000, -1.000000000000000000 ) ) ;
#119854=EDGE_LOOP ( 'NONE', ( #99851, #91440 ) ) ;
#119855=AXIS2_PLACEMENT_3D ( 'NONE', #48808, #30463, #119449 ) ;
#119856=ORIENTED_EDGE ( 'NONE', *, *, #85888, .F. ) ;
#119857=DIRECTION ( 'NONE',  ( -0.000000000000000000, 1.000000000000000000, -0.000000000000000000 ) ) ;
#119858=ORIENTED_EDGE ( 'NONE', *, *, #90194, .F. ) ;
#119859=CARTESIAN_POINT ( 'NONE',  ( -9.999999999999969802, 12.50000000000000000, -2.276824562219559311E-15 ) ) ;
#119860=ORIENTED_EDGE ( 'NONE', *, *, #108587, .F. ) ;
#119861=ADVANCED_FACE ( 'NONE', ( #65245 ), #85460, .T. ) ;
#119862=EDGE_CURVE ( 'NONE', #93340, #110466, #127249, .T. ) ;
#119863=ORIENTED_EDGE ( 'NONE', *, *, #65688, .F. ) ;
#119864=DIRECTION ( 'NONE',  ( -0.000000000000000000, -1.000000000000000000, -0.000000000000000000 ) ) ;
#119865=DIRECTION ( 'NONE',  ( -4.274815082592931898E-19, -0.9999939076577903929, -0.003490651415223739937 ) ) ;
#119866=DIRECTION ( 'NONE',  ( 0.000000000000000000, 0.000000000000000000, 1.000000000000000000 ) ) ;
#119867=DIRECTION ( 'NONE',  ( -0.000000000000000000, 1.000000000000000000, -0.000000000000000000 ) ) ;
#119868=CARTESIAN_POINT ( 'NONE',  ( 17.50000000000000000, 0.4166666666666649088, 4.000000000000000888 ) ) ;
#119869=VERTEX_POINT ( 'NONE', #5683 ) ;
#119870=DIRECTION ( 'NONE',  ( 0.000000000000000000, 1.000000000000000000, 0.000000000000000000 ) ) ;
#119871=DIRECTION ( 'NONE',  ( 0.000000000000000000, -0.9999939076577903929, 0.003490651415223739937 ) ) ;
#119872=AXIS2_PLACEMENT_3D ( 'NONE', #73959, #113889, #102760 ) ;
#119873=AXIS2_PLACEMENT_3D ( 'NONE', #58651, #78942, #109011 ) ;
#119874=EDGE_CURVE ( 'NONE', #16094, #8551, #72955, .T. ) ;
#119875=CARTESIAN_POINT ( 'NONE',  ( -8.950000000000009948, 12.50000000000000000, 2.511473670974873507 ) ) ;
#119876=FACE_OUTER_BOUND ( 'NONE', #105382, .T. ) ;
#119877=DIRECTION ( 'NONE',  ( 0.000000000000000000, 0.000000000000000000, -1.000000000000000000 ) ) ;
#119878=VERTEX_POINT ( 'NONE', #50151 ) ;
#119879=AXIS2_PLACEMENT_3D ( 'NONE', #37000, #126668, #8165 ) ;
#119880=CONICAL_SURFACE ( 'NONE', #80172, 0.09999999999999982514, 0.003490658503988666988 ) ;
#119881=AXIS2_PLACEMENT_3D ( 'NONE', #18838, #26735, #58140 ) ;
#119882=ORIENTED_EDGE ( 'NONE', *, *, #81357, .T. ) ;
#119883=CIRCLE ( 'NONE', #107352, 0.06509327318403745899 ) ;
#119884=AXIS2_PLACEMENT_3D ( 'NONE', #99108, #88632, #49375 ) ;
#119885=CARTESIAN_POINT ( 'NONE',  ( 2.499999999999947153, 2.500000000000000000, -3.737306695894649700 ) ) ;
#119886=ORIENTED_EDGE ( 'NONE', *, *, #93776, .F. ) ;
#119887=DIRECTION ( 'NONE',  ( -4.274815082592931898E-19, -0.9999939076577903929, -0.003490651415223739937 ) ) ;
#119889=CONICAL_SURFACE ( 'NONE', #57195, 0.1000000000000002554, 0.003490658503988666988 ) ;
#119890=CIRCLE ( 'NONE', #13265, 0.06509327318403745899 ) ;
#119891=VECTOR ( 'NONE', #99663, 1000.000000000000000 ) ;
#119892=AXIS2_PLACEMENT_3D ( 'NONE', #46910, #86817, #105821 ) ;
#119893=CONICAL_SURFACE ( 'NONE', #80102, 0.09999999999999999167, 0.003490658503988666988 ) ;
#119896=DIRECTION ( 'NONE',  ( -0.000000000000000000, 1.000000000000000000, -0.000000000000000000 ) ) ;
#119897=CARTESIAN_POINT ( 'NONE',  ( 3.349999999999941913, 2.500000000000000000, 5.802370205355744659 ) ) ;
#119898=DIRECTION ( 'NONE',  ( 0.000000000000000000, 1.000000000000000000, 0.000000000000000000 ) ) ;
#119899=EDGE_CURVE ( 'NONE', #73855, #121027, #78968, .T. ) ;
#119900=CARTESIAN_POINT ( 'NONE',  ( 4.149999999999939959, 2.500000000000000000, -6.495190528383302464 ) ) ;
#119901=EDGE_LOOP ( 'NONE', ( #129181, #30749 ) ) ;
#119902=EDGE_CURVE ( 'NONE', #56812, #70717, #10256, .T. ) ;
#119903=CARTESIAN_POINT ( 'NONE',  ( 43.06183256894050260, 3.066944586325434319, -4.904925618674059962 ) ) ;
#119904=CARTESIAN_POINT ( 'NONE',  ( 7.099999999999928590, 12.50000000000000000, 3.637306695894644726 ) ) ;
#119905=EDGE_CURVE ( 'NONE', #69440, #70666, #104252, .T. ) ;
#119906=CARTESIAN_POINT ( 'NONE',  ( -8.350000000000008527, 2.500000000000000000, 7.088010851410848190 ) ) ;
#119907=AXIS2_PLACEMENT_3D ( 'NONE', #51189, #1418, #19108 ) ;
#119908=ORIENTED_EDGE ( 'NONE', *, *, #57458, .T. ) ;
#119909=EDGE_CURVE ( 'NONE', #32951, #92601, #368, .T. ) ;
#119910=ADVANCED_FACE ( 'NONE', ( #30522 ), #100053, .T. ) ;
#119911=ORIENTED_EDGE ( 'NONE', *, *, #73303, .F. ) ;
#119912=LINE ( 'NONE', #51827, #50179 ) ;
#119913=DIRECTION ( 'NONE',  ( 0.000000000000000000, 0.000000000000000000, 1.000000000000000000 ) ) ;
#119914=EDGE_CURVE ( 'NONE', #108686, #16687, #75007, .T. ) ;
#119915=CARTESIAN_POINT ( 'NONE',  ( 12.69999999999990337, 2.500000000000000000, -4.576537180435978236 ) ) ;
#119916=CONICAL_SURFACE ( 'NONE', #23781, 0.1000000000000002554, 0.003490658503988666988 ) ;
#119917=VERTEX_POINT ( 'NONE', #129370 ) ;
#119918=AXIS2_PLACEMENT_3D ( 'NONE', #66953, #106882, #107549 ) ;
#119919=VECTOR ( 'NONE', #55989, 1000.000000000000000 ) ;
#119920=CARTESIAN_POINT ( 'NONE',  ( 5.399999999999936406, 12.50000000000000000, -3.637306695894650055 ) ) ;
#119921=EDGE_CURVE ( 'NONE', #57691, #13400, #59988, .T. ) ;
#119922=CARTESIAN_POINT ( 'NONE',  ( 12.69999999999989804, 2.500000000000000000, 0.3464101615137735735 ) ) ;
#119923=ORIENTED_EDGE ( 'NONE', *, *, #26637, .F. ) ;
#119924=CARTESIAN_POINT ( 'NONE',  ( -10.40000000000000213, 2.500000000000000000, 4.330127018922196314 ) ) ;
#119925=AXIS2_PLACEMENT_3D ( 'NONE', #39146, #99976, #29946 ) ;
#119926=ORIENTED_EDGE ( 'NONE', *, *, #44132, .F. ) ;
#119927=CIRCLE ( 'NONE', #63501, 0.06509327318403745899 ) ;
#119928=ADVANCED_FACE ( 'NONE', ( #10214 ), #40330, .T. ) ;
#119929=CARTESIAN_POINT ( 'NONE',  ( 6.449999999999930012, 2.500000000000000000, 6.841600689897072485 ) ) ;
#119930=AXIS2_PLACEMENT_3D ( 'NONE', #90016, #70398, #21288 ) ;
#119931=AXIS2_PLACEMENT_3D ( 'NONE', #14736, #75605, #44889 ) ;
#119932=EDGE_LOOP ( 'NONE', ( #69297, #68811, #10203, #32103 ) ) ;
#119933=DIRECTION ( 'NONE',  ( 0.000000000000000000, 1.000000000000000000, 0.000000000000000000 ) ) ;
#119934=DIRECTION ( 'NONE',  ( 0.000000000000000000, 0.000000000000000000, 1.000000000000000000 ) ) ;
#119935=ORIENTED_EDGE ( 'NONE', *, *, #23366, .F. ) ;
#119936=ORIENTED_EDGE ( 'NONE', *, *, #7245, .T. ) ;
#119937=AXIS2_PLACEMENT_3D ( 'NONE', #125438, #35773, #47530 ) ;
#119938=DIRECTION ( 'NONE',  ( -0.000000000000000000, -1.000000000000000000, -0.000000000000000000 ) ) ;
#119939=DIRECTION ( 'NONE',  ( 0.000000000000000000, 0.000000000000000000, -1.000000000000000000 ) ) ;
#119940=EDGE_LOOP ( 'NONE', ( #106155, #66488 ) ) ;
#119941=DIRECTION ( 'NONE',  ( -0.000000000000000000, -1.000000000000000000, -0.000000000000000000 ) ) ;
#119943=AXIS2_PLACEMENT_3D ( 'NONE', #36860, #46037, #126525 ) ;
#119944=DIRECTION ( 'NONE',  ( 0.000000000000000000, 0.000000000000000000, 1.000000000000000000 ) ) ;
#119945=AXIS2_PLACEMENT_3D ( 'NONE', #129355, #86816, #109019 ) ;
#119947=DIRECTION ( 'NONE',  ( -0.000000000000000000, 1.000000000000000000, -0.000000000000000000 ) ) ;
#119948=DIRECTION ( 'NONE',  ( 0.000000000000000000, 0.000000000000000000, 1.000000000000000000 ) ) ;
#119949=AXIS2_PLACEMENT_3D ( 'NONE', #125888, #36252, #76171 ) ;
#119950=CARTESIAN_POINT ( 'NONE',  ( 1.649999999999950617, 2.500000000000000000, -2.265063509461101798 ) ) ;
#119951=CIRCLE ( 'NONE', #2882, 0.09999999999999982514 ) ;
#119952=EDGE_LOOP ( 'NONE', ( #62112, #33080 ) ) ;
#119953=VERTEX_POINT ( 'NONE', #109711 ) ;
#119954=ORIENTED_EDGE ( 'NONE', *, *, #42787, .F. ) ;
#119955=CARTESIAN_POINT ( 'NONE',  ( -14.34999999999998543, 12.50000000000000000, -2.511473670974875727 ) ) ;
#119956=CARTESIAN_POINT ( 'NONE',  ( -0.6500000000000394351, 12.50000000000000000, 2.511473670974873507 ) ) ;
#119957=DIRECTION ( 'NONE',  ( 0.000000000000000000, 0.000000000000000000, 1.000000000000000000 ) ) ;
#119958=EDGE_LOOP ( 'NONE', ( #52649, #78882, #117232, #33504 ) ) ;
#119959=VERTEX_POINT ( 'NONE', #69775 ) ;
#119960=FACE_BOUND ( 'NONE', #14459, .T. ) ;
#119961=EDGE_LOOP ( 'NONE', ( #34722, #33124 ) ) ;
#119962=CARTESIAN_POINT ( 'NONE',  ( -0.4000000000000392131, 2.500000000000000000, -5.022947341949754119 ) ) ;
#119963=CARTESIAN_POINT ( 'NONE',  ( 14.99999999999989164, 2.500000000000000000, 0.5928203230275495006 ) ) ;
#119964=LINE ( 'NONE', #30316, #36737 ) ;
#119965=EDGE_CURVE ( 'NONE', #126837, #73054, #20044, .T. ) ;
#119966=CARTESIAN_POINT ( 'NONE',  ( -12.89999999999999325, 2.500000000000000000, -3.737306695894647035 ) ) ;
#119967=DIRECTION ( 'NONE',  ( -0.000000000000000000, 1.000000000000000000, -0.000000000000000000 ) ) ;
#119968=DIRECTION ( 'NONE',  ( -0.000000000000000000, -1.000000000000000000, -0.000000000000000000 ) ) ;
#119969=CARTESIAN_POINT ( 'NONE',  ( -7.499999999999976907, 2.500000000000000000, 4.430127018922196847 ) ) ;
#119970=CIRCLE ( 'NONE', #2894, 0.1000000000000000472 ) ;
#119971=DIRECTION ( 'NONE',  ( 0.000000000000000000, 1.000000000000000000, 0.000000000000000000 ) ) ;
#119972=CARTESIAN_POINT ( 'NONE',  ( 14.39999999999989555, 2.500000000000000000, -0.3464101615137782364 ) ) ;
#119973=EDGE_CURVE ( 'NONE', #97481, #126422, #70796, .T. ) ;
#119974=AXIS2_PLACEMENT_3D ( 'NONE', #50062, #100427, #10724 ) ;
#119975=CIRCLE ( 'NONE', #86511, 0.09999999999999982514 ) ;
#119976=EDGE_LOOP ( 'NONE', ( #31471, #28581, #88362, #95700 ) ) ;
#119977=ORIENTED_EDGE ( 'NONE', *, *, #111957, .T. ) ;
#119978=ORIENTED_EDGE ( 'NONE', *, *, #28497, .T. ) ;
#119979=ORIENTED_EDGE ( 'NONE', *, *, #77983, .F. ) ;
#119980=LINE ( 'NONE', #100345, #22814 ) ;
#119981=VECTOR ( 'NONE', #42906, 1000.000000000000000 ) ;
#119982=AXIS2_PLACEMENT_3D ( 'NONE', #1372, #61611, #31493 ) ;
#119983=CARTESIAN_POINT ( 'NONE',  ( 9.349999999999916156, 2.500000000000000000, 6.841600689897072485 ) ) ;
#119984=ORIENTED_EDGE ( 'NONE', *, *, #101281, .F. ) ;
#119985=EDGE_LOOP ( 'NONE', ( #124117, #97128, #63742, #54670 ) ) ;
#119986=ORIENTED_EDGE ( 'NONE', *, *, #48427, .F. ) ;
#119987=CARTESIAN_POINT ( 'NONE',  ( 7.699999999999925571, 12.50000000000000000, 3.983716857408420076 ) ) ;
#119988=VECTOR ( 'NONE', #84310, 1000.000000000000000 ) ;
#119989=CIRCLE ( 'NONE', #15406, 0.06509327318403741736 ) ;
#119990=CONICAL_SURFACE ( 'NONE', #36474, 0.1000000000000002554, 0.003490658503988666988 ) ;
#119991=FACE_OUTER_BOUND ( 'NONE', #30850, .T. ) ;
#119992=CARTESIAN_POINT ( 'NONE',  ( 9.149999999999916866, 2.500000000000000000, -2.957883832488653830 ) ) ;
#119993=DIRECTION ( 'NONE',  ( 0.000000000000000000, 1.000000000000000000, 0.000000000000000000 ) ) ;
#119994=FACE_OUTER_BOUND ( 'NONE', #55064, .T. ) ;
#119996=CIRCLE ( 'NONE', #9173, 0.1000000000000002554 ) ;
#119997=DIRECTION ( 'NONE',  ( -4.274815082592931898E-19, -0.9999939076577903929, -0.003490651415223739937 ) ) ;
#119998=ORIENTED_EDGE ( 'NONE', *, *, #106428, .F. ) ;
#119999=CARTESIAN_POINT ( 'NONE',  ( 5.649999999999934630, 2.500000000000000000, 6.148780366869520897 ) ) ;
#120000=VERTEX_POINT ( 'NONE', #48201 ) ;
#120001=VERTEX_POINT ( 'NONE', #69122 ) ;
#120002=ORIENTED_EDGE ( 'NONE', *, *, #18673, .F. ) ;
#120003=CIRCLE ( 'NONE', #17574, 0.09999999999999982514 ) ;
#120004=DIRECTION ( 'NONE',  ( 0.000000000000000000, 0.000000000000000000, -1.000000000000000000 ) ) ;
#120005=VERTEX_POINT ( 'NONE', #58035 ) ;
#120006=ORIENTED_EDGE ( 'NONE', *, *, #36483, .F. ) ;
#120007=CIRCLE ( 'NONE', #17579, 0.1000000000000002554 ) ;
#120009=EDGE_CURVE ( 'NONE', #74917, #122022, #91727, .T. ) ;
#120010=DIRECTION ( 'NONE',  ( 0.000000000000000000, 1.000000000000000000, 0.000000000000000000 ) ) ;
#120011=DIRECTION ( 'NONE',  ( 0.000000000000000000, 0.000000000000000000, -1.000000000000000000 ) ) ;
#120012=CARTESIAN_POINT ( 'NONE',  ( 3.349999999999943689, 2.500000000000000000, 2.165063509461097713 ) ) ;
#120013=DIRECTION ( 'NONE',  ( 0.000000000000000000, -0.000000000000000000, 1.000000000000000000 ) ) ;
#120014=EDGE_LOOP ( 'NONE', ( #64340, #16672 ) ) ;
#120015=CARTESIAN_POINT ( 'NONE',  ( 9.799999999999913669, 2.500000000000000000, -3.883716857408426648 ) ) ;
#120016=AXIS2_PLACEMENT_3D ( 'NONE', #9674, #69889, #39801 ) ;
#120017=ADVANCED_FACE ( 'NONE', ( #29224 ), #20638, .T. ) ;
#120019=ORIENTED_EDGE ( 'NONE', *, *, #122019, .T. ) ;
#120020=CARTESIAN_POINT ( 'NONE',  ( 16.55712542097768392, -0.2763552092527354342, 6.093697598458595266 ) ) ;
#120021=EDGE_LOOP ( 'NONE', ( #118084, #25390, #111732, #7247 ) ) ;
#120023=CARTESIAN_POINT ( 'NONE',  ( -9.600000000000008527, 12.50000000000000000, -3.637306695894645614 ) ) ;
#120024=ORIENTED_EDGE ( 'NONE', *, *, #40794, .F. ) ;
#120025=FACE_OUTER_BOUND ( 'NONE', #114767, .T. ) ;
#120026=EDGE_CURVE ( 'NONE', #11005, #3528, #37364, .T. ) ;
#120027=DIRECTION ( 'NONE',  ( 0.000000000000000000, -0.000000000000000000, 1.000000000000000000 ) ) ;
#120028=AXIS2_PLACEMENT_3D ( 'NONE', #8199, #81471, #31721 ) ;
#120029=EDGE_CURVE ( 'NONE', #61538, #48101, #24830, .T. ) ;
#120030=ORIENTED_EDGE ( 'NONE', *, *, #67693, .T. ) ;
#120031=CONICAL_SURFACE ( 'NONE', #15543, 0.1000000000000002554, 0.003490658503988666988 ) ;
#120032=ADVANCED_FACE ( 'NONE', ( #108404 ), #110509, .T. ) ;
#120033=LINE ( 'NONE', #63041, #34225 ) ;
#120034=EDGE_LOOP ( 'NONE', ( #13434, #43955, #72817, #7014 ) ) ;
#120035=ORIENTED_EDGE ( 'NONE', *, *, #82880, .T. ) ;
#120036=DIRECTION ( 'NONE',  ( 0.000000000000000000, 0.000000000000000000, 1.000000000000000000 ) ) ;
#120037=CARTESIAN_POINT ( 'NONE',  ( -0.8500000000000386136, 2.500000000000000000, 7.188010851410848723 ) ) ;
#120038=EDGE_CURVE ( 'NONE', #30034, #12327, #54074, .T. ) ;
#120039=LINE ( 'NONE', #118738, #125335 ) ;
#120040=DIRECTION ( 'NONE',  ( 0.000000000000000000, 1.000000000000000000, 0.000000000000000000 ) ) ;
#120041=CARTESIAN_POINT ( 'NONE',  ( -10.65000000000000213, 12.50000000000000000, 6.083687093685482772 ) ) ;
#120042=EDGE_LOOP ( 'NONE', ( #111484, #65469 ) ) ;
#120043=CIRCLE ( 'NONE', #32422, 0.06509327318403745899 ) ;
#120044=AXIS2_PLACEMENT_3D ( 'NONE', #1653, #11483, #119269 ) ;
#120045=DIRECTION ( 'NONE',  ( -0.000000000000000000, -1.000000000000000000, -0.000000000000000000 ) ) ;
#120046=CONICAL_SURFACE ( 'NONE', #101255, 0.1000000000000000472, 0.003490658503988666988 ) ;
#120047=VERTEX_POINT ( 'NONE', #109033 ) ;
#120048=CIRCLE ( 'NONE', #17624, 0.09999999999999999167 ) ;
#120049=CARTESIAN_POINT ( 'NONE',  ( 7.699999999999925571, 2.500000000000000000, 3.983716857408420076 ) ) ;
#120050=CARTESIAN_POINT ( 'NONE',  ( 4.149999999999941735, 12.50000000000000000, -1.472243186433550122 ) ) ;
#120052=DIRECTION ( 'NONE',  ( 0.000000000000000000, 0.000000000000000000, 1.000000000000000000 ) ) ;
#120053=CARTESIAN_POINT ( 'NONE',  ( 1.649999999999951061, 12.50000000000000000, -6.495190528383302464 ) ) ;
#120054=FACE_OUTER_BOUND ( 'NONE', #42116, .T. ) ;
#120055=CARTESIAN_POINT ( 'NONE',  ( 11.84999999999990727, 12.50000000000000000, 6.213873640053558134 ) ) ;
#120056=ORIENTED_EDGE ( 'NONE', *, *, #30876, .T. ) ;
#120057=DIRECTION ( 'NONE',  ( 0.000000000000000000, 0.000000000000000000, 1.000000000000000000 ) ) ;
#120058=CIRCLE ( 'NONE', #63630, 0.06509327318403745899 ) ;
#120059=FACE_OUTER_BOUND ( 'NONE', #40712, .T. ) ;
#120060=DIRECTION ( 'NONE',  ( 0.000000000000000000, 1.000000000000000000, 0.000000000000000000 ) ) ;
#120061=AXIS2_PLACEMENT_3D ( 'NONE', #38750, #30692, #6635 ) ;
#120062=CIRCLE ( 'NONE', #120152, 0.06509327318403745899 ) ;
#120063=CONICAL_SURFACE ( 'NONE', #11387, 0.1000000000000002554, 0.003490658503988666988 ) ;
#120064=VERTEX_POINT ( 'NONE', #59340 ) ;
#120065=ADVANCED_FACE ( 'NONE', ( #104833 ), #81269, .T. ) ;
#120066=CARTESIAN_POINT ( 'NONE',  ( 3.349999999999945466, 12.50000000000000000, -7.188010851410854052 ) ) ;
#120068=AXIS2_PLACEMENT_3D ( 'NONE', #9075, #58198, #50953 ) ;
#120069=VERTEX_POINT ( 'NONE', #96305 ) ;
#120070=CIRCLE ( 'NONE', #40675, 0.1000000000000002554 ) ;
#120071=ORIENTED_EDGE ( 'NONE', *, *, #112691, .F. ) ;
#120072=CARTESIAN_POINT ( 'NONE',  ( 2.899999999999943956, 2.500000000000000000, 4.330127018922196314 ) ) ;
#120073=ADVANCED_FACE ( 'NONE', ( #15813 ), #95040, .T. ) ;
#120074=ORIENTED_EDGE ( 'NONE', *, *, #80307, .T. ) ;
#120075=CARTESIAN_POINT ( 'NONE',  ( 12.89999999999989910, 2.500000000000000000, -0.6928203230275542523 ) ) ;
#120076=DIRECTION ( 'NONE',  ( -0.000000000000000000, -1.000000000000000000, -0.000000000000000000 ) ) ;
#120077=ADVANCED_FACE ( 'NONE', ( #15153 ), #104343, .T. ) ;
#120078=EDGE_CURVE ( 'NONE', #73868, #49718, #45303, .T. ) ;
#120079=VECTOR ( 'NONE', #45690, 1000.000000000000000 ) ;
#120080=VERTEX_POINT ( 'NONE', #16447 ) ;
#120081=CIRCLE ( 'NONE', #40680, 0.1000000000000000472 ) ;
#120082=AXIS2_PLACEMENT_3D ( 'NONE', #64085, #15613, #33985 ) ;
#120083=DIRECTION ( 'NONE',  ( -0.000000000000000000, -1.000000000000000000, -0.000000000000000000 ) ) ;
#120084=EDGE_CURVE ( 'NONE', #34772, #74521, #6126, .T. ) ;
#120085=CARTESIAN_POINT ( 'NONE',  ( 3.749999999999944045, 12.50000000000000000, -2.792790559304616504 ) ) ;
#120086=AXIS2_PLACEMENT_3D ( 'NONE', #43104, #63361, #83016 ) ;
#120087=DIRECTION ( 'NONE',  ( 0.000000000000000000, 0.000000000000000000, -1.000000000000000000 ) ) ;
#120088=ORIENTED_EDGE ( 'NONE', *, *, #53147, .F. ) ;
#120089=ADVANCED_FACE ( 'NONE', ( #75376 ), #41672, .T. ) ;
#120090=ADVANCED_FACE ( 'NONE', ( #66845 ), #29142, .T. ) ;
#120091=ORIENTED_EDGE ( 'NONE', *, *, #27775, .F. ) ;
#120092=VERTEX_POINT ( 'NONE', #26301 ) ;
#120093=DIRECTION ( 'NONE',  ( 0.000000000000000000, 1.000000000000000000, 0.000000000000000000 ) ) ;
#120094=FACE_OUTER_BOUND ( 'NONE', #88452, .T. ) ;
#120095=DIRECTION ( 'NONE',  ( 0.000000000000000000, 1.000000000000000000, 0.000000000000000000 ) ) ;
#120096=FACE_BOUND ( 'NONE', #32084, .T. ) ;
#120097=EDGE_LOOP ( 'NONE', ( #50343, #74078 ) ) ;
#120098=DIRECTION ( 'NONE',  ( 0.000000000000000000, 0.000000000000000000, 1.000000000000000000 ) ) ;
#120099=CARTESIAN_POINT ( 'NONE',  ( 8.749999999999953815, 2.500000000000000000, 6.395190528383296602 ) ) ;
#120100=AXIS2_PLACEMENT_3D ( 'NONE', #106190, #25045, #64954 ) ;
#120101=VERTEX_POINT ( 'NONE', #17745 ) ;
#120102=CARTESIAN_POINT ( 'NONE',  ( -6.650000000000014566, 2.500000000000000000, 6.395190528383296602 ) ) ;
#120103=DIRECTION ( 'NONE',  ( -0.000000000000000000, 1.000000000000000000, -0.000000000000000000 ) ) ;
#120104=CARTESIAN_POINT ( 'NONE',  ( 0.3999999999999568345, 2.500000000000000000, -3.537306695894649966 ) ) ;
#120105=CARTESIAN_POINT ( 'NONE',  ( 14.54999999999989235, 12.50000000000000000, -2.165063509461101710 ) ) ;
#120106=DIRECTION ( 'NONE',  ( -0.000000000000000000, 1.000000000000000000, -0.000000000000000000 ) ) ;
#120107=CARTESIAN_POINT ( 'NONE',  ( 2.699999999999947331, 2.500000000000000000, -0.3464101615137783474 ) ) ;
#120108=EDGE_CURVE ( 'NONE', #111656, #115693, #121064, .T. ) ;
#120109=DIRECTION ( 'NONE',  ( -0.000000000000000000, -1.000000000000000000, -0.000000000000000000 ) ) ;
#120110=ORIENTED_EDGE ( 'NONE', *, *, #86940, .F. ) ;
#120111=ORIENTED_EDGE ( 'NONE', *, *, #113779, .F. ) ;
#120112=ORIENTED_EDGE ( 'NONE', *, *, #50319, .T. ) ;
#120113=VERTEX_POINT ( 'NONE', #85207 ) ;
#120114=CARTESIAN_POINT ( 'NONE',  ( 5.449999999999936229, 2.500000000000000000, 6.395190528383296602 ) ) ;
#120115=DIRECTION ( 'NONE',  ( 0.000000000000000000, -0.000000000000000000, 1.000000000000000000 ) ) ;
#120116=EDGE_CURVE ( 'NONE', #35149, #9410, #110596, .T. ) ;
#120117=EDGE_LOOP ( 'NONE', ( #93044, #116347, #35353, #14779 ) ) ;
#120118=FACE_BOUND ( 'NONE', #109210, .T. ) ;
#120119=DIRECTION ( 'NONE',  ( 0.000000000000000000, 1.000000000000000000, 0.000000000000000000 ) ) ;
#120120=CIRCLE ( 'NONE', #97129, 0.06509327318403745899 ) ;
#120121=LINE ( 'NONE', #51398, #120267 ) ;
#120123=AXIS2_PLACEMENT_3D ( 'NONE', #24315, #5304, #64237 ) ;
#120124=DIRECTION ( 'NONE',  ( -0.000000000000000000, -1.000000000000000000, -0.000000000000000000 ) ) ;
#120125=CARTESIAN_POINT ( 'NONE',  ( -1.850000000000033396, 12.50000000000000000, -1.753560074763288457 ) ) ;
#120126=DIRECTION ( 'NONE',  ( 0.000000000000000000, -0.9999939076577903929, 0.003490651415223739937 ) ) ;
#120127=DIRECTION ( 'NONE',  ( 0.000000000000000000, 1.000000000000000000, 0.000000000000000000 ) ) ;
#120128=ORIENTED_EDGE ( 'NONE', *, *, #120029, .T. ) ;
#120129=EDGE_LOOP ( 'NONE', ( #52329, #56011, #82, #54249 ) ) ;
#120130=ADVANCED_FACE ( 'NONE', ( #25633 ), #27076, .T. ) ;
#120131=AXIS2_PLACEMENT_3D ( 'NONE', #17686, #69362, #47812 ) ;
#120132=ORIENTED_EDGE ( 'NONE', *, *, #56090, .F. ) ;
#120133=ORIENTED_EDGE ( 'NONE', *, *, #45750, .T. ) ;
#120134=AXIS2_PLACEMENT_3D ( 'NONE', #59287, #49466, #67787 ) ;
#120135=VERTEX_POINT ( 'NONE', #47231 ) ;
#120136=ORIENTED_EDGE ( 'NONE', *, *, #13938, .T. ) ;
#120137=DIRECTION ( 'NONE',  ( 0.000000000000000000, 0.000000000000000000, 1.000000000000000000 ) ) ;
#120138=CARTESIAN_POINT ( 'NONE',  ( -7.300000000000018474, 12.50000000000000000, -3.983716857408426293 ) ) ;
#120139=CIRCLE ( 'NONE', #118068, 0.09999999999999982514 ) ;
#120140=ORIENTED_EDGE ( 'NONE', *, *, #109392, .F. ) ;
#120141=CARTESIAN_POINT ( 'NONE',  ( 4.999999999999935163, 12.50000000000000000, 3.637306695894644726 ) ) ;
#120142=CARTESIAN_POINT ( 'NONE',  ( -3.550000000000027800, 2.500000000000000000, 6.248780366869520542 ) ) ;
#120144=CARTESIAN_POINT ( 'NONE',  ( 6.449999999999931788, 12.50000000000000000, 6.148780366869520009 ) ) ;
#120145=CARTESIAN_POINT ( 'NONE',  ( -9.600000000000006750, 2.500000000000000000, -0.6928203230275542523 ) ) ;
#120146=EDGE_LOOP ( 'NONE', ( #75050, #51262 ) ) ;
#120147=DIRECTION ( 'NONE',  ( 0.000000000000000000, 0.000000000000000000, -1.000000000000000000 ) ) ;
#120148=ORIENTED_EDGE ( 'NONE', *, *, #96914, .T. ) ;
#120149=VECTOR ( 'NONE', #95552, 1000.000000000000000 ) ;
#120150=EDGE_LOOP ( 'NONE', ( #99424, #58997 ) ) ;
#120151=CARTESIAN_POINT ( 'NONE',  ( -7.100000000000017408, 2.500000000000000000, -0.7928203230275543412 ) ) ;
#120152=AXIS2_PLACEMENT_3D ( 'NONE', #81538, #71713, #103758 ) ;
#120153=PLANE ( 'NONE',  #88644 ) ;
#120154=CIRCLE ( 'NONE', #59549, 0.1000000000000000472 ) ;
#120155=DIRECTION ( 'NONE',  ( -0.000000000000000000, -1.000000000000000000, -0.000000000000000000 ) ) ;
#120156=ORIENTED_EDGE ( 'NONE', *, *, #106338, .F. ) ;
#120157=VERTEX_POINT ( 'NONE', #105505 ) ;
#120158=CARTESIAN_POINT ( 'NONE',  ( -5.450000000000019718, 12.50000000000000000, 6.495190528383297135 ) ) ;
#120159=AXIS2_PLACEMENT_3D ( 'NONE', #88096, #110194, #60471 ) ;
#120160=AXIS2_PLACEMENT_3D ( 'NONE', #29354, #117047, #67286 ) ;
#120161=CIRCLE ( 'NONE', #95122, 0.06509327318403745899 ) ;
#120162=DIRECTION ( 'NONE',  ( -0.000000000000000000, -1.000000000000000000, -0.000000000000000000 ) ) ;
#120163=CARTESIAN_POINT ( 'NONE',  ( -12.09999999999999609, 2.500000000000000000, -4.922947341949750921 ) ) ;
#120164=CARTESIAN_POINT ( 'NONE',  ( 12.89999999999989733, 2.500000000000000000, 0.09999999999999761857 ) ) ;
#120165=ORIENTED_EDGE ( 'NONE', *, *, #99194, .T. ) ;
#120166=CIRCLE ( 'NONE', #19917, 0.09999999999999982514 ) ;
#120167=CARTESIAN_POINT ( 'NONE',  ( -5.650000000000023448, 2.500000000000000000, -6.841600689897078702 ) ) ;
#120168=ORIENTED_EDGE ( 'NONE', *, *, #85868, .T. ) ;
#120170=AXIS2_PLACEMENT_3D ( 'NONE', #106496, #38422, #67178 ) ;
#120171=CIRCLE ( 'NONE', #84660, 0.09999999999999982514 ) ;
#120173=ORIENTED_EDGE ( 'NONE', *, *, #99237, .F. ) ;
#120174=CARTESIAN_POINT ( 'NONE',  ( -11.69999999999999929, 2.500000000000000000, 1.734723475976807094E-15 ) ) ;
#120175=DIRECTION ( 'NONE',  ( -0.000000000000000000, 1.000000000000000000, -0.000000000000000000 ) ) ;
#120176=DIRECTION ( 'NONE',  ( 0.000000000000000000, 0.000000000000000000, 1.000000000000000000 ) ) ;
#120177=AXIS2_PLACEMENT_3D ( 'NONE', #78349, #71092, #51466 ) ;
#120178=ADVANCED_FACE ( 'NONE', ( #45945 ), #24923, .T. ) ;
#120179=DIRECTION ( 'NONE',  ( 0.000000000000000000, 1.000000000000000000, 0.000000000000000000 ) ) ;
#120180=EDGE_CURVE ( 'NONE', #98287, #54837, #50077, .T. ) ;
#120181=EDGE_LOOP ( 'NONE', ( #55699, #89492, #58283, #19914 ) ) ;
#120182=DIRECTION ( 'NONE',  ( 0.000000000000000000, 0.000000000000000000, 1.000000000000000000 ) ) ;
#120183=ADVANCED_FACE ( 'NONE', ( #27557 ), #54177, .T. ) ;
#120184=DIRECTION ( 'NONE',  ( 0.000000000000000000, 0.000000000000000000, 1.000000000000000000 ) ) ;
#120186=EDGE_CURVE ( 'NONE', #91471, #124289, #45855, .T. ) ;
#120187=ORIENTED_EDGE ( 'NONE', *, *, #52665, .F. ) ;
#120188=EDGE_CURVE ( 'NONE', #121037, #16096, #39618, .T. ) ;
#120189=ORIENTED_EDGE ( 'NONE', *, *, #80516, .F. ) ;
#120190=DIRECTION ( 'NONE',  ( 0.000000000000000000, -0.000000000000000000, 1.000000000000000000 ) ) ;
#120191=DIRECTION ( 'NONE',  ( 0.000000000000000000, 0.000000000000000000, -1.000000000000000000 ) ) ;
#120192=CARTESIAN_POINT ( 'NONE',  ( -4.600000000000025402, 2.500000000000000000, -2.385244779468109755E-15 ) ) ;
#120193=ADVANCED_FACE ( 'NONE', ( #108712 ), #119007, .T. ) ;
#120194=DIRECTION ( 'NONE',  ( 0.000000000000000000, 1.000000000000000000, 0.000000000000000000 ) ) ;
#120195=CIRCLE ( 'NONE', #7297, 0.09999999999999999167 ) ;
#120196=CARTESIAN_POINT ( 'NONE',  ( -1.450000000000035483, 2.500000000000000000, 1.818653347947321475 ) ) ;
#120197=DIRECTION ( 'NONE',  ( -0.000000000000000000, -1.000000000000000000, -0.000000000000000000 ) ) ;
#120198=DIRECTION ( 'NONE',  ( 0.000000000000000000, -0.9999939076577903929, 0.003490651415223739937 ) ) ;
#120199=DIRECTION ( 'NONE',  ( -0.000000000000000000, 1.000000000000000000, -0.000000000000000000 ) ) ;
#120200=FACE_OUTER_BOUND ( 'NONE', #2585, .T. ) ;
#120201=EDGE_CURVE ( 'NONE', #125681, #54589, #100193, .T. ) ;
#120202=AXIS2_PLACEMENT_3D ( 'NONE', #112239, #61203, #52664 ) ;
#120203=AXIS2_PLACEMENT_3D ( 'NONE', #67246, #114444, #24790 ) ;
#120205=DIRECTION ( 'NONE',  ( -0.000000000000000000, -1.000000000000000000, -0.000000000000000000 ) ) ;
#120206=DIRECTION ( 'NONE',  ( -0.000000000000000000, 1.000000000000000000, -0.000000000000000000 ) ) ;
#120207=CARTESIAN_POINT ( 'NONE',  ( -2.100000000000033840, 2.500000000000000000, 3.737306695894644371 ) ) ;
#120208=CARTESIAN_POINT ( 'NONE',  ( 3.349999999999941913, 12.50000000000000000, 6.560283801567334372 ) ) ;
#120209=CARTESIAN_POINT ( 'NONE',  ( 2.099999999999948574, 2.500000000000000000, 3.737306695894644371 ) ) ;
#120210=EDGE_LOOP ( 'NONE', ( #21269, #80527 ) ) ;
#120211=CARTESIAN_POINT ( 'NONE',  ( -1.450000000000035039, 2.500000000000000000, -6.741600689897077281 ) ) ;
#120212=CIRCLE ( 'NONE', #15727, 0.06509327318403745899 ) ;
#120213=VECTOR ( 'NONE', #67945, 1000.000000000000000 ) ;
#120214=DIRECTION ( 'NONE',  ( 0.000000000000000000, 1.000000000000000000, 0.000000000000000000 ) ) ;
#120215=DIRECTION ( 'NONE',  ( 0.000000000000000000, 0.000000000000000000, -1.000000000000000000 ) ) ;
#120216=VERTEX_POINT ( 'NONE', #8560 ) ;
#120217=ADVANCED_FACE ( 'NONE', ( #39991 ), #2206, .T. ) ;
#120218=VERTEX_POINT ( 'NONE', #60900 ) ;
#120219=DIRECTION ( 'NONE',  ( 0.000000000000000000, 1.000000000000000000, 0.000000000000000000 ) ) ;
#120220=AXIS2_PLACEMENT_3D ( 'NONE', #123312, #32392, #72297 ) ;
#120221=VECTOR ( 'NONE', #123341, 1000.000000000000000 ) ;
#120222=EDGE_LOOP ( 'NONE', ( #10413, #27169 ) ) ;
#120223=ORIENTED_EDGE ( 'NONE', *, *, #113389, .F. ) ;
#120224=DIRECTION ( 'NONE',  ( 0.000000000000000000, 1.000000000000000000, 0.000000000000000000 ) ) ;
#120225=EDGE_CURVE ( 'NONE', #119487, #47194, #118528, .T. ) ;
#120226=EDGE_CURVE ( 'NONE', #121748, #125596, #9232, .T. ) ;
#120227=CARTESIAN_POINT ( 'NONE',  ( 18.37149739119586656, 2.540880845002003063, -2.596776292461022706 ) ) ;
#120228=DIRECTION ( 'NONE',  ( -0.000000000000000000, 1.000000000000000000, -0.000000000000000000 ) ) ;
#120229=EDGE_CURVE ( 'NONE', #78481, #114814, #47921, .T. ) ;
#120230=FACE_OUTER_BOUND ( 'NONE', #35471, .T. ) ;
#120231=ORIENTED_EDGE ( 'NONE', *, *, #121287, .F. ) ;
#120232=ADVANCED_FACE ( 'NONE', ( #49817 ), #16583, .T. ) ;
#120234=EDGE_LOOP ( 'NONE', ( #126819, #16618, #63071, #123408 ) ) ;
#120235=DIRECTION ( 'NONE',  ( 0.000000000000000000, 1.000000000000000000, 0.000000000000000000 ) ) ;
#120236=ADVANCED_FACE ( 'NONE', ( #19029 ), #687, .T. ) ;
#120237=DIRECTION ( 'NONE',  ( 0.000000000000000000, 1.000000000000000000, 0.000000000000000000 ) ) ;
#120238=ADVANCED_FACE ( 'NONE', ( #89719 ), #89084, .T. ) ;
#120239=DIRECTION ( 'NONE',  ( 0.000000000000000000, 0.000000000000000000, 1.000000000000000000 ) ) ;
#120240=ADVANCED_FACE ( 'NONE', ( #47879 ), #29518, .T. ) ;
#120241=ORIENTED_EDGE ( 'NONE', *, *, #67786, .F. ) ;
#120242=ADVANCED_FACE ( 'NONE', ( #77961 ), #109356, .T. ) ;
#120243=EDGE_CURVE ( 'NONE', #105724, #33641, #8182, .T. ) ;
#120244=AXIS2_PLACEMENT_3D ( 'NONE', #23419, #93462, #92164 ) ;
#120245=VERTEX_POINT ( 'NONE', #82495 ) ;
#120246=VERTEX_POINT ( 'NONE', #71352 ) ;
#120247=CONICAL_SURFACE ( 'NONE', #97249, 0.09999999999999982514, 0.003490658503988666988 ) ;
#120248=ORIENTED_EDGE ( 'NONE', *, *, #60804, .T. ) ;
#120249=ORIENTED_EDGE ( 'NONE', *, *, #97425, .F. ) ;
#120250=CARTESIAN_POINT ( 'NONE',  ( -14.14999999999998614, 12.50000000000000000, 2.165063509461101265 ) ) ;
#120251=CARTESIAN_POINT ( 'NONE',  ( 10.30524027349397898, 1.500000000000000222, 9.130939513664273477 ) ) ;
#120252=AXIS2_PLACEMENT_3D ( 'NONE', #60285, #97597, #100186 ) ;
#120253=DIRECTION ( 'NONE',  ( 0.000000000000000000, 0.000000000000000000, 1.000000000000000000 ) ) ;
#120254=FACE_BOUND ( 'NONE', #20515, .T. ) ;
#120255=LINE ( 'NONE', #60695, #124597 ) ;
#120257=EDGE_CURVE ( 'NONE', #100851, #26800, #70901, .T. ) ;
#120258=FACE_OUTER_BOUND ( 'NONE', #8183, .T. ) ;
#120259=CARTESIAN_POINT ( 'NONE',  ( -7.950000000000012612, 2.500000000000000000, 2.165063509461097713 ) ) ;
#120260=AXIS2_PLACEMENT_3D ( 'NONE', #62679, #12893, #122882 ) ;
#120261=AXIS2_PLACEMENT_3D ( 'NONE', #31637, #21828, #82684 ) ;
#120262=DIRECTION ( 'NONE',  ( -0.000000000000000000, -1.000000000000000000, -0.000000000000000000 ) ) ;
#120263=AXIS2_PLACEMENT_3D ( 'NONE', #60023, #10868, #90745 ) ;
#120264=FACE_OUTER_BOUND ( 'NONE', #16459, .T. ) ;
#120265=LINE ( 'NONE', #10909, #19859 ) ;
#120266=CIRCLE ( 'NONE', #84753, 0.06509327318403745899 ) ;
#120267=VECTOR ( 'NONE', #21261, 1000.000000000000000 ) ;
#120268=CARTESIAN_POINT ( 'NONE',  ( 5.799999999999931433, 2.500000000000000000, 4.430127018922196847 ) ) ;
#120269=VERTEX_POINT ( 'NONE', #122415 ) ;
#120270=ORIENTED_EDGE ( 'NONE', *, *, #10123, .T. ) ;
#120271=ORIENTED_EDGE ( 'NONE', *, *, #57729, .T. ) ;
#120272=ORIENTED_EDGE ( 'NONE', *, *, #106727, .F. ) ;
#120273=AXIS2_PLACEMENT_3D ( 'NONE', #17792, #7327, #68181 ) ;
#120274=DIRECTION ( 'NONE',  ( -4.274815082592931898E-19, -0.9999939076577903929, -0.003490651415223739937 ) ) ;
#120275=DIRECTION ( 'NONE',  ( 0.000000000000000000, 0.000000000000000000, 1.000000000000000000 ) ) ;
#120276=FACE_BOUND ( 'NONE', #30708, .T. ) ;
#120277=CARTESIAN_POINT ( 'NONE',  ( 1.049999999999954969, 2.500000000000000000, -6.841600689897077814 ) ) ;
#120278=VERTEX_POINT ( 'NONE', #52373 ) ;
#120279=DIRECTION ( 'NONE',  ( -0.000000000000000000, -1.000000000000000000, -0.000000000000000000 ) ) ;
#120280=DIRECTION ( 'NONE',  ( 0.000000000000000000, 0.000000000000000000, -1.000000000000000000 ) ) ;
#120281=FACE_OUTER_BOUND ( 'NONE', #67099, .T. ) ;
#120282=DIRECTION ( 'NONE',  ( 0.000000000000000000, 0.000000000000000000, 1.000000000000000000 ) ) ;
#120283=AXIS2_PLACEMENT_3D ( 'NONE', #126397, #85178, #15122 ) ;
#120284=VERTEX_POINT ( 'NONE', #2611 ) ;
#120285=LINE ( 'NONE', #30627, #74329 ) ;
#120286=ADVANCED_FACE ( 'NONE', ( #64122 ), #33356, .T. ) ;
#120287=ORIENTED_EDGE ( 'NONE', *, *, #87733, .F. ) ;
#120288=EDGE_LOOP ( 'NONE', ( #115080, #14316 ) ) ;
#120289=DIRECTION ( 'NONE',  ( 0.000000000000000000, -0.000000000000000000, 1.000000000000000000 ) ) ;
#120290=CARTESIAN_POINT ( 'NONE',  ( -7.950000000000016165, 2.500000000000000000, -6.595190528383296780 ) ) ;
#120292=AXIS2_PLACEMENT_3D ( 'NONE', #25780, #105644, #86634 ) ;
#120295=FACE_OUTER_BOUND ( 'NONE', #106230, .T. ) ;
#120296=CARTESIAN_POINT ( 'NONE',  ( 2.899999999999946620, 12.50000000000000000, -5.022947341949754119 ) ) ;
#120297=VERTEX_POINT ( 'NONE', #103414 ) ;
#120298=ADVANCED_FACE ( 'NONE', ( #32761 ), #92957, .T. ) ;
#120299=DIRECTION ( 'NONE',  ( 0.000000000000000000, 0.000000000000000000, 1.000000000000000000 ) ) ;
#120300=ORIENTED_EDGE ( 'NONE', *, *, #7628, .T. ) ;
#120301=DIRECTION ( 'NONE',  ( 0.000000000000000000, 1.000000000000000000, 0.000000000000000000 ) ) ;
#120302=VECTOR ( 'NONE', #59723, 1000.000000000000000 ) ;
#120303=EDGE_LOOP ( 'NONE', ( #75005, #17045, #81465, #32009 ) ) ;
#120304=CIRCLE ( 'NONE', #1165, 0.06509327318403745899 ) ;
#120305=CARTESIAN_POINT ( 'NONE',  ( 1.649999999999949729, 2.500000000000000000, 5.802370205355744659 ) ) ;
#120306=VERTEX_POINT ( 'NONE', #83140 ) ;
#120307=CARTESIAN_POINT ( 'NONE',  ( 5.849999999999933920, 2.500000000000000000, -2.857883832488653741 ) ) ;
#120308=CARTESIAN_POINT ( 'NONE',  ( -1.250000000000001110, 2.500000000000000000, -2.265063509461101798 ) ) ;
#120309=CARTESIAN_POINT ( 'NONE',  ( 11.04999999999991012, 12.50000000000000000, 6.841600689897072485 ) ) ;
#120310=CARTESIAN_POINT ( 'NONE',  ( -3.150000000000033218, 12.50000000000000000, -6.841600689897078702 ) ) ;
#120311=DIRECTION ( 'NONE',  ( 0.000000000000000000, 1.000000000000000000, 0.000000000000000000 ) ) ;
#120312=EDGE_LOOP ( 'NONE', ( #89772, #85784, #26550, #120995 ) ) ;
#120313=ORIENTED_EDGE ( 'NONE', *, *, #78347, .T. ) ;
#120314=ORIENTED_EDGE ( 'NONE', *, *, #39420, .T. ) ;
#120315=DIRECTION ( 'NONE',  ( 0.000000000000000000, 1.000000000000000000, 0.000000000000000000 ) ) ;
#120316=CIRCLE ( 'NONE', #3328, 0.1000000000000002554 ) ;
#120317=VECTOR ( 'NONE', #127220, 1000.000000000000000 ) ;
#120318=DIRECTION ( 'NONE',  ( 0.000000000000000000, 0.000000000000000000, -1.000000000000000000 ) ) ;
#120320=VERTEX_POINT ( 'NONE', #1332 ) ;
#120321=ORIENTED_EDGE ( 'NONE', *, *, #105605, .T. ) ;
#120322=ORIENTED_EDGE ( 'NONE', *, *, #33169, .F. ) ;
#120323=DIRECTION ( 'NONE',  ( 0.000000000000000000, -0.9999939076577903929, 0.003490651415223739937 ) ) ;
#120324=ORIENTED_EDGE ( 'NONE', *, *, #32557, .T. ) ;
#120325=DIRECTION ( 'NONE',  ( 0.000000000000000000, 0.000000000000000000, -1.000000000000000000 ) ) ;
#120326=EDGE_CURVE ( 'NONE', #93646, #1061, #68831, .T. ) ;
#120327=CARTESIAN_POINT ( 'NONE',  ( -14.14999999999998614, 2.500000000000000000, 2.165063509461101265 ) ) ;
#120328=CARTESIAN_POINT ( 'NONE',  ( -0.2000000000000408673, 2.500000000000000000, -4.083716857408426826 ) ) ;
#120329=AXIS2_PLACEMENT_3D ( 'NONE', #44311, #94064, #73764 ) ;
#120330=DIRECTION ( 'NONE',  ( 0.000000000000000000, 1.000000000000000000, 0.000000000000000000 ) ) ;
#120333=AXIS2_PLACEMENT_3D ( 'NONE', #11656, #51601, #30028 ) ;
#120334=CARTESIAN_POINT ( 'NONE',  ( -11.05000000000000071, 2.500000000000000000, -2.411473670974874306 ) ) ;
#120335=EDGE_CURVE ( 'NONE', #3627, #107815, #66764, .T. ) ;
#120336=ORIENTED_EDGE ( 'NONE', *, *, #44107, .F. ) ;
#120337=ORIENTED_EDGE ( 'NONE', *, *, #107806, .T. ) ;
#120338=LINE ( 'NONE', #20203, #119732 ) ;
#120339=AXIS2_PLACEMENT_3D ( 'NONE', #43510, #44134, #55252 ) ;
#120340=AXIS2_PLACEMENT_3D ( 'NONE', #58398, #59699, #57749 ) ;
#120341=FACE_OUTER_BOUND ( 'NONE', #125484, .T. ) ;
#120342=EDGE_CURVE ( 'NONE', #66203, #35924, #75100, .T. ) ;
#120343=ORIENTED_EDGE ( 'NONE', *, *, #67446, .F. ) ;
#120344=ADVANCED_FACE ( 'NONE', ( #1973 ), #24208, .T. ) ;
#120345=ORIENTED_EDGE ( 'NONE', *, *, #52462, .F. ) ;
#120346=EDGE_CURVE ( 'NONE', #39511, #126455, #108544, .T. ) ;
#120348=CARTESIAN_POINT ( 'NONE',  ( 1.849999999999949685, 12.50000000000000000, 1.818653347947321475 ) ) ;
#120349=EDGE_CURVE ( 'NONE', #98829, #74234, #41285, .T. ) ;
#120350=EDGE_CURVE ( 'NONE', #51798, #81523, #31022, .T. ) ;
#120351=DIRECTION ( 'NONE',  ( 0.000000000000000000, 0.000000000000000000, 1.000000000000000000 ) ) ;
#120352=CIRCLE ( 'NONE', #21871, 0.09999999999999982514 ) ;
#120353=CARTESIAN_POINT ( 'NONE',  ( -6.250000000000019540, 12.50000000000000000, -7.188010851410854052 ) ) ;
#120354=DIRECTION ( 'NONE',  ( -0.000000000000000000, 1.000000000000000000, -0.000000000000000000 ) ) ;
#120355=CARTESIAN_POINT ( 'NONE',  ( -2.950000000000029932, 2.500000000000000000, -2.065063509461102065 ) ) ;
#120356=DIRECTION ( 'NONE',  ( 0.000000000000000000, 1.000000000000000000, 0.000000000000000000 ) ) ;
#120357=ADVANCED_FACE ( 'NONE', ( #3913 ), #102094, .T. ) ;
#120358=DIRECTION ( 'NONE',  ( 0.000000000000000000, 0.000000000000000000, 1.000000000000000000 ) ) ;
#120359=EDGE_CURVE ( 'NONE', #115626, #122432, #120866, .T. ) ;
#120360=VERTEX_POINT ( 'NONE', #111266 ) ;
#120361=EDGE_CURVE ( 'NONE', #69008, #24259, #4077, .T. ) ;
#120362=ORIENTED_EDGE ( 'NONE', *, *, #90949, .T. ) ;
#120363=CONICAL_SURFACE ( 'NONE', #80651, 0.09999999999999982514, 0.003490658503988666988 ) ;
#120364=VERTEX_POINT ( 'NONE', #11799 ) ;
#120365=ORIENTED_EDGE ( 'NONE', *, *, #99399, .T. ) ;
#120366=EDGE_LOOP ( 'NONE', ( #54288, #79519, #110792, #85524 ) ) ;
#120367=DIRECTION ( 'NONE',  ( 0.000000000000000000, -0.9999939076577903929, 0.003490651415223739937 ) ) ;
#120368=DIRECTION ( 'NONE',  ( 0.000000000000000000, 0.000000000000000000, 1.000000000000000000 ) ) ;
#120369=ORIENTED_EDGE ( 'NONE', *, *, #87402, .T. ) ;
#120370=DIRECTION ( 'NONE',  ( -0.000000000000000000, 1.000000000000000000, -0.000000000000000000 ) ) ;
#120371=CARTESIAN_POINT ( 'NONE',  ( 1.649999999999950617, 2.500000000000000000, -2.165063509461101710 ) ) ;
#120372=CARTESIAN_POINT ( 'NONE',  ( 12.09999999999990195, 2.500000000000000000, -0.7928203230275542301 ) ) ;
#120373=DIRECTION ( 'NONE',  ( 0.000000000000000000, 0.000000000000000000, 1.000000000000000000 ) ) ;
#120374=EDGE_LOOP ( 'NONE', ( #85489, #53610, #81943, #33983 ) ) ;
#120375=CARTESIAN_POINT ( 'NONE',  ( 0.5999999999999551248, 2.500000000000000000, -4.676537180435978769 ) ) ;
#120376=AXIS2_PLACEMENT_3D ( 'NONE', #107241, #45759, #115774 ) ;
#120377=PLANE ( 'NONE',  #91717 ) ;
#120378=VERTEX_POINT ( 'NONE', #51740 ) ;
#120380=ORIENTED_EDGE ( 'NONE', *, *, #40847, .T. ) ;
#120381=VERTEX_POINT ( 'NONE', #91652 ) ;
#120383=AXIS2_PLACEMENT_3D ( 'NONE', #121089, #22268, #120448 ) ;
#120384=AXIS2_PLACEMENT_3D ( 'NONE', #127200, #115394, #85948 ) ;
#120385=DIRECTION ( 'NONE',  ( -0.000000000000000000, -1.000000000000000000, -0.000000000000000000 ) ) ;
#120386=CARTESIAN_POINT ( 'NONE',  ( -3.750000000000026201, 12.50000000000000000, 5.802370205355744659 ) ) ;
#120387=AXIS2_PLACEMENT_3D ( 'NONE', #54562, #56501, #96418 ) ;
#120388=DIRECTION ( 'NONE',  ( 0.000000000000000000, -0.9999939076577903929, 0.003490651415223739937 ) ) ;
#120389=ORIENTED_EDGE ( 'NONE', *, *, #95807, .T. ) ;
#120390=DIRECTION ( 'NONE',  ( -4.274815082592931898E-19, -0.9999939076577903929, -0.003490651415223739937 ) ) ;
#120391=CARTESIAN_POINT ( 'NONE',  ( -3.150000000000030109, 12.50000000000000000, 1.818653347947321475 ) ) ;
#120392=CARTESIAN_POINT ( 'NONE',  ( -9.150000000000009237, 12.50000000000000000, 2.165063509461097713 ) ) ;
#120393=DIRECTION ( 'NONE',  ( 0.000000000000000000, 0.000000000000000000, 1.000000000000000000 ) ) ;
#120394=EDGE_CURVE ( 'NONE', #79468, #44082, #62214, .T. ) ;
#120395=AXIS2_PLACEMENT_3D ( 'NONE', #89012, #20908, #58268 ) ;
#120396=EDGE_CURVE ( 'NONE', #62169, #18680, #68640, .T. ) ;
#120397=VERTEX_POINT ( 'NONE', #7122 ) ;
#120398=DIRECTION ( 'NONE',  ( 0.000000000000000000, 0.000000000000000000, -1.000000000000000000 ) ) ;
#120399=CIRCLE ( 'NONE', #66008, 0.06509327318403745899 ) ;
#120400=VECTOR ( 'NONE', #20483, 1000.000000000000000 ) ;
#120401=ADVANCED_FACE ( 'NONE', ( #64762 ), #62401, .T. ) ;
#120402=ORIENTED_EDGE ( 'NONE', *, *, #77347, .F. ) ;
#120403=ORIENTED_EDGE ( 'NONE', *, *, #24749, .F. ) ;
#120404=CARTESIAN_POINT ( 'NONE',  ( 1.649999999999951061, 2.500000000000000000, -6.495190528383302464 ) ) ;
#120405=CARTESIAN_POINT ( 'NONE',  ( 0.3999999999999619971, 12.50000000000000000, 0.06509327318403732021 ) ) ;
#120406=FACE_BOUND ( 'NONE', #11410, .T. ) ;
#120407=DIRECTION ( 'NONE',  ( 0.000000000000000000, 1.000000000000000000, 0.000000000000000000 ) ) ;
#120408=DIRECTION ( 'NONE',  ( 0.000000000000000000, 0.000000000000000000, -1.000000000000000000 ) ) ;
#120409=EDGE_CURVE ( 'NONE', #72896, #101165, #5920, .T. ) ;
#120410=DIRECTION ( 'NONE',  ( 0.000000000000000000, 1.000000000000000000, 0.000000000000000000 ) ) ;
#120411=VECTOR ( 'NONE', #11934, 1000.000000000000000 ) ;
#120412=CARTESIAN_POINT ( 'NONE',  ( -5.850000000000021849, 12.50000000000000000, -1.472243186433550122 ) ) ;
#120413=DIRECTION ( 'NONE',  ( 0.000000000000000000, -0.9999939076577903929, 0.003490651415223739937 ) ) ;
#120414=FACE_OUTER_BOUND ( 'NONE', #19101, .T. ) ;
#120415=ORIENTED_EDGE ( 'NONE', *, *, #100692, .T. ) ;
#120416=CARTESIAN_POINT ( 'NONE',  ( -14.54999999999998472, 2.500000000000000000, 2.165063509461101265 ) ) ;
#120417=DIRECTION ( 'NONE',  ( -4.274815082592931898E-19, -0.9999939076577903929, -0.003490651415223739937 ) ) ;
#120418=VERTEX_POINT ( 'NONE', #37260 ) ;
#120419=VERTEX_POINT ( 'NONE', #55596 ) ;
#120420=CARTESIAN_POINT ( 'NONE',  ( 13.54999999999989591, 2.500000000000000000, -1.818653347947326138 ) ) ;
#120422=EDGE_CURVE ( 'NONE', #119869, #100266, #20811, .T. ) ;
#120423=FACE_BOUND ( 'NONE', #61923, .T. ) ;
#120424=CARTESIAN_POINT ( 'NONE',  ( 11.24999999999990763, 12.50000000000000000, 1.472243186433545459 ) ) ;
#120425=CIRCLE ( 'NONE', #11753, 0.09999999999999982514 ) ;
#120426=DIRECTION ( 'NONE',  ( -0.000000000000000000, -1.000000000000000000, -0.000000000000000000 ) ) ;
#120427=AXIS2_PLACEMENT_3D ( 'NONE', #21029, #80609, #81868 ) ;
#120428=ORIENTED_EDGE ( 'NONE', *, *, #105752, .T. ) ;
#120429=CARTESIAN_POINT ( 'NONE',  ( 87.49999999944498086, 3.974992050012154277, 6.359987280019447020 ) ) ;
#120431=ORIENTED_EDGE ( 'NONE', *, *, #83395, .F. ) ;
#120432=PLANE ( 'NONE',  #21892 ) ;
#120434=AXIS2_PLACEMENT_3D ( 'NONE', #68358, #128611, #67711 ) ;
#120435=AXIS2_PLACEMENT_3D ( 'NONE', #50874, #71807, #9658 ) ;
#120436=EDGE_CURVE ( 'NONE', #51752, #29463, #58486, .T. ) ;
#120437=DIRECTION ( 'NONE',  ( 0.000000000000000000, 0.000000000000000000, 1.000000000000000000 ) ) ;
#120438=DIRECTION ( 'NONE',  ( -0.000000000000000000, -1.000000000000000000, -0.000000000000000000 ) ) ;
#120439=VECTOR ( 'NONE', #47927, 1000.000000000000000 ) ;
#120440=VERTEX_POINT ( 'NONE', #77171 ) ;
#120441=AXIS2_PLACEMENT_3D ( 'NONE', #96962, #28236, #68142 ) ;
#120442=CARTESIAN_POINT ( 'NONE',  ( -7.100000000000013856, 12.50000000000000000, 3.572213422710607489 ) ) ;
#120443=CARTESIAN_POINT ( 'NONE',  ( -10.20000000000000639, 2.500000000000000000, -4.083716857408422385 ) ) ;
#120444=FACE_OUTER_BOUND ( 'NONE', #128934, .T. ) ;
#120445=ORIENTED_EDGE ( 'NONE', *, *, #127592, .T. ) ;
#120446=ORIENTED_EDGE ( 'NONE', *, *, #52106, .F. ) ;
#120447=EDGE_CURVE ( 'NONE', #7522, #126712, #56860, .T. ) ;
#120448=DIRECTION ( 'NONE',  ( 0.000000000000000000, 0.000000000000000000, -1.000000000000000000 ) ) ;
#120449=EDGE_LOOP ( 'NONE', ( #84203, #111907 ) ) ;
#120450=DIRECTION ( 'NONE',  ( 0.000000000000000000, -0.000000000000000000, 1.000000000000000000 ) ) ;
#120451=CARTESIAN_POINT ( 'NONE',  ( 17.50000000000000000, -2.499999999999999556, 0.6666666666666717367 ) ) ;
#120452=DIRECTION ( 'NONE',  ( 0.000000000000000000, 0.000000000000000000, 1.000000000000000000 ) ) ;
#120453=ORIENTED_EDGE ( 'NONE', *, *, #111630, .T. ) ;
#120454=CARTESIAN_POINT ( 'NONE',  ( 6.249999999999967137, 2.500000000000000000, -2.065063509461102065 ) ) ;
#120455=DIRECTION ( 'NONE',  ( 0.000000000000000000, 0.000000000000000000, 1.000000000000000000 ) ) ;
#120456=DIRECTION ( 'NONE',  ( -0.000000000000000000, 1.000000000000000000, -0.000000000000000000 ) ) ;
#120457=CARTESIAN_POINT ( 'NONE',  ( -11.05000000000000071, 2.500000000000000000, -6.841600689897075149 ) ) ;
#120459=DIRECTION ( 'NONE',  ( 0.000000000000000000, -0.000000000000000000, 1.000000000000000000 ) ) ;
#120460=VERTEX_POINT ( 'NONE', #94226 ) ;
#120461=ORIENTED_EDGE ( 'NONE', *, *, #52211, .T. ) ;
#120462=CARTESIAN_POINT ( 'NONE',  ( 11.64999999999990266, 2.500000000000000000, -6.495190528383302464 ) ) ;
#120463=VERTEX_POINT ( 'NONE', #46408 ) ;
#120464=CONICAL_SURFACE ( 'NONE', #1326, 0.09999999999999999167, 0.003490658503988666988 ) ;
#120466=ORIENTED_EDGE ( 'NONE', *, *, #57148, .T. ) ;
#120467=EDGE_LOOP ( 'NONE', ( #105341, #89618, #44779, #87930 ) ) ;
#120468=AXIS2_PLACEMENT_3D ( 'NONE', #66030, #48331, #58169 ) ;
#120470=DIRECTION ( 'NONE',  ( 0.000000000000000000, 0.000000000000000000, 1.000000000000000000 ) ) ;
#120471=CIRCLE ( 'NONE', #30606, 0.06509327318403745899 ) ;
#120472=AXIS2_PLACEMENT_3D ( 'NONE', #100311, #42032, #52481 ) ;
#120473=CARTESIAN_POINT ( 'NONE',  ( -11.84999999999999609, 12.50000000000000000, 6.841600689897072485 ) ) ;
#120474=DIRECTION ( 'NONE',  ( 0.000000000000000000, 0.000000000000000000, 1.000000000000000000 ) ) ;
#120475=AXIS2_PLACEMENT_3D ( 'NONE', #43171, #14313, #24800 ) ;
#120476=EDGE_CURVE ( 'NONE', #23253, #98415, #98160, .T. ) ;
#120478=CARTESIAN_POINT ( 'NONE',  ( -6.650000000000018119, 12.50000000000000000, -2.922977105672691422 ) ) ;
#120479=LINE ( 'NONE', #81829, #6199 ) ;
#120480=CARTESIAN_POINT ( 'NONE',  ( -1.450000000000035039, 2.500000000000000000, -6.841600689897077814 ) ) ;
#120481=DIRECTION ( 'NONE',  ( -0.000000000000000000, -1.000000000000000000, -0.000000000000000000 ) ) ;
#120482=DIRECTION ( 'NONE',  ( -0.000000000000000000, -1.000000000000000000, -0.000000000000000000 ) ) ;
#120483=PLANE ( 'NONE',  #95846 ) ;
#120484=AXIS2_PLACEMENT_3D ( 'NONE', #19459, #128805, #39776 ) ;
#120485=ADVANCED_FACE ( 'NONE', ( #104679 ), #104148, .T. ) ;
#120486=ORIENTED_EDGE ( 'NONE', *, *, #54768, .F. ) ;
#120487=CIRCLE ( 'NONE', #53596, 0.1000000000000002554 ) ;
#120488=CIRCLE ( 'NONE', #11813, 0.06509327318403745899 ) ;
#120489=CARTESIAN_POINT ( 'NONE',  ( 10.59999999999990905, 2.500000000000000000, -4.676537180435978769 ) ) ;
#120490=ADVANCED_FACE ( 'NONE', ( #105985 ), #7990, .T. ) ;
#120491=VERTEX_POINT ( 'NONE', #96157 ) ;
#120492=EDGE_CURVE ( 'NONE', #58724, #34741, #76960, .T. ) ;
#120493=VERTEX_POINT ( 'NONE', #26780 ) ;
#120494=ADVANCED_FACE ( 'NONE', ( #26144 ), #110683, .T. ) ;
#120495=CARTESIAN_POINT ( 'NONE',  ( 5.799999999999933209, 2.500000000000000000, 0.09999999999999761857 ) ) ;
#120496=ADVANCED_FACE ( 'NONE', ( #4528 ), #70982, .T. ) ;
#120497=DIRECTION ( 'NONE',  ( 0.000000000000000000, 0.000000000000000000, -1.000000000000000000 ) ) ;
#120498=CARTESIAN_POINT ( 'NONE',  ( -12.49999999999999289, 2.500000000000000000, -5.022947341949751454 ) ) ;
#120499=DIRECTION ( 'NONE',  ( 0.000000000000000000, 0.000000000000000000, 1.000000000000000000 ) ) ;
#120500=DIRECTION ( 'NONE',  ( 0.000000000000000000, 1.000000000000000000, 0.000000000000000000 ) ) ;
#120501=EDGE_CURVE ( 'NONE', #84780, #80574, #104430, .T. ) ;
#120502=CARTESIAN_POINT ( 'NONE',  ( -10.00000000000000355, 2.500000000000000000, 3.537306695894645081 ) ) ;
#120503=ORIENTED_EDGE ( 'NONE', *, *, #121181, .T. ) ;
#120504=EDGE_CURVE ( 'NONE', #26800, #100851, #54262, .T. ) ;
#120505=ADVANCED_FACE ( 'NONE', ( #66054 ), #31292, .T. ) ;
#120506=EDGE_CURVE ( 'NONE', #85926, #4878, #48013, .T. ) ;
#120507=ORIENTED_EDGE ( 'NONE', *, *, #10512, .F. ) ;
#120508=CARTESIAN_POINT ( 'NONE',  ( 16.56576425165006228, 2.500000000000000444, -6.084390597445811011 ) ) ;
#120509=EDGE_CURVE ( 'NONE', #42494, #65236, #125607, .T. ) ;
#120510=ORIENTED_EDGE ( 'NONE', *, *, #35993, .T. ) ;
#120511=CARTESIAN_POINT ( 'NONE',  ( 9.149999999999920419, 2.500000000000000000, 1.572243186433545548 ) ) ;
#120512=ORIENTED_EDGE ( 'NONE', *, *, #117667, .F. ) ;
#120513=ORIENTED_EDGE ( 'NONE', *, *, #74726, .T. ) ;
#120514=EDGE_CURVE ( 'NONE', #86064, #72341, #93683, .T. ) ;
#120515=PLANE ( 'NONE',  #4314 ) ;
#120516=DIRECTION ( 'NONE',  ( 0.000000000000000000, 1.000000000000000000, 0.000000000000000000 ) ) ;
#120517=CONICAL_SURFACE ( 'NONE', #24374, 0.1000000000000002554, 0.003490658503988666988 ) ;
#120518=CARTESIAN_POINT ( 'NONE',  ( -7.100000000000014744, 12.50000000000000000, 4.265033745738159077 ) ) ;
#120519=CIRCLE ( 'NONE', #22331, 0.09999999999999982514 ) ;
#120520=LINE ( 'NONE', #110685, #19631 ) ;
#120521=CARTESIAN_POINT ( 'NONE',  ( -9.600000000000008527, 2.500000000000000000, -4.922947341949749145 ) ) ;
#120522=VERTEX_POINT ( 'NONE', #18243 ) ;
#120524=DIRECTION ( 'NONE',  ( 0.000000000000000000, 0.000000000000000000, -1.000000000000000000 ) ) ;
#120525=DIRECTION ( 'NONE',  ( -0.000000000000000000, -1.000000000000000000, -0.000000000000000000 ) ) ;
#120526=DIRECTION ( 'NONE',  ( 0.000000000000000000, 1.000000000000000000, 0.000000000000000000 ) ) ;
#120527=DIRECTION ( 'NONE',  ( 0.000000000000000000, 1.000000000000000000, 0.000000000000000000 ) ) ;
#120528=AXIS2_PLACEMENT_3D ( 'NONE', #60349, #108771, #51810 ) ;
#120529=CIRCLE ( 'NONE', #103799, 0.1000000000000000472 ) ;
#120530=DIRECTION ( 'NONE',  ( 0.000000000000000000, 0.000000000000000000, 1.000000000000000000 ) ) ;
#120531=VERTEX_POINT ( 'NONE', #127561 ) ;
#120532=VERTEX_POINT ( 'NONE', #129525 ) ;
#120533=CARTESIAN_POINT ( 'NONE',  ( -5.600000000000020073, 12.50000000000000000, -0.3464101615137782364 ) ) ;
#120534=ORIENTED_EDGE ( 'NONE', *, *, #35579, .F. ) ;
#120535=AXIS2_PLACEMENT_3D ( 'NONE', #44586, #95619, #104765 ) ;
#120536=DIRECTION ( 'NONE',  ( 0.000000000000000000, 0.000000000000000000, -1.000000000000000000 ) ) ;
#120537=DIRECTION ( 'NONE',  ( 0.000000000000000000, 0.000000000000000000, 1.000000000000000000 ) ) ;
#120538=CONICAL_SURFACE ( 'NONE', #47385, 0.09999999999999982514, 0.003490658503988666988 ) ;
#120539=ORIENTED_EDGE ( 'NONE', *, *, #5526, .F. ) ;
#120540=CARTESIAN_POINT ( 'NONE',  ( -8.350000000000013856, 2.500000000000000000, -5.902370205355745192 ) ) ;
#120541=DIRECTION ( 'NONE',  ( 0.000000000000000000, 0.000000000000000000, -1.000000000000000000 ) ) ;
#120542=DIRECTION ( 'NONE',  ( 0.000000000000000000, 0.000000000000000000, 1.000000000000000000 ) ) ;
#120543=DIRECTION ( 'NONE',  ( 0.000000000000000000, 0.000000000000000000, 1.000000000000000000 ) ) ;
#120544=EDGE_CURVE ( 'NONE', #23954, #87583, #85367, .T. ) ;
#120545=CARTESIAN_POINT ( 'NONE',  ( -0.8000000000000381251, 12.50000000000000000, 4.265033745738159077 ) ) ;
#120546=EDGE_CURVE ( 'NONE', #68963, #68394, #53978, .T. ) ;
#120547=ORIENTED_EDGE ( 'NONE', *, *, #117075, .F. ) ;
#120548=CARTESIAN_POINT ( 'NONE',  ( 76.45352548353409361, 3.568407488302709041, -6.085611496483662286 ) ) ;
#120549=CIRCLE ( 'NONE', #126813, 0.06509327318403745899 ) ;
#120550=DIRECTION ( 'NONE',  ( 0.000000000000000000, 0.000000000000000000, 1.000000000000000000 ) ) ;
#120551=CARTESIAN_POINT ( 'NONE',  ( -2.900000000000029221, 12.50000000000000000, -0.7579135962115916003 ) ) ;
#120552=AXIS2_PLACEMENT_3D ( 'NONE', #175, #98377, #108845 ) ;
#120553=EDGE_CURVE ( 'NONE', #45205, #17761, #9070, .T. ) ;
#120554=CARTESIAN_POINT ( 'NONE',  ( 11.64999999999990621, 2.500000000000000000, -2.265063509461101798 ) ) ;
#120555=VERTEX_POINT ( 'NONE', #90189 ) ;
#120556=CIRCLE ( 'NONE', #1415, 0.06509327318403745899 ) ;
#120557=VERTEX_POINT ( 'NONE', #118376 ) ;
#120559=DIRECTION ( 'NONE',  ( 0.000000000000000000, 0.000000000000000000, 1.000000000000000000 ) ) ;
#120560=AXIS2_PLACEMENT_3D ( 'NONE', #27218, #107720, #68431 ) ;
#120561=CARTESIAN_POINT ( 'NONE',  ( 7.699999999999925571, 2.500000000000000000, -4.576537180435978236 ) ) ;
#120562=AXIS2_PLACEMENT_3D ( 'NONE', #34147, #35440, #77753 ) ;
#120563=ORIENTED_EDGE ( 'NONE', *, *, #59932, .T. ) ;
#120564=CARTESIAN_POINT ( 'NONE',  ( 8.949999999999915801, 2.500000000000000000, -1.918653347947326004 ) ) ;
#120565=VECTOR ( 'NONE', #71417, 1000.000000000000000 ) ;
#120566=CARTESIAN_POINT ( 'NONE',  ( 7.949999999999922018, 2.500000000000000000, -2.165063509461101710 ) ) ;
#120567=ORIENTED_EDGE ( 'NONE', *, *, #37299, .T. ) ;
#120568=CARTESIAN_POINT ( 'NONE',  ( 4.399999999999940847, 12.50000000000000000, -4.741630453620015118 ) ) ;
#120569=AXIS2_PLACEMENT_3D ( 'NONE', #90335, #129027, #99548 ) ;
#120570=VERTEX_POINT ( 'NONE', #87622 ) ;
#120571=CARTESIAN_POINT ( 'NONE',  ( -6.050000000000018474, 2.500000000000000000, 6.741600689897071952 ) ) ;
#120572=CIRCLE ( 'NONE', #51635, 0.1000000000000002554 ) ;
#120573=AXIS2_PLACEMENT_3D ( 'NONE', #55578, #6435, #116414 ) ;
#120574=EDGE_LOOP ( 'NONE', ( #33138, #102600, #98380, #3057 ) ) ;
#120575=DIRECTION ( 'NONE',  ( -4.274815082592931898E-19, -0.9999939076577903929, -0.003490651415223739937 ) ) ;
#120576=DIRECTION ( 'NONE',  ( -0.000000000000000000, -1.000000000000000000, -0.000000000000000000 ) ) ;
#120577=ORIENTED_EDGE ( 'NONE', *, *, #64781, .T. ) ;
#120578=ORIENTED_EDGE ( 'NONE', *, *, #21012, .T. ) ;
#120579=DIRECTION ( 'NONE',  ( 0.000000000000000000, 0.000000000000000000, -1.000000000000000000 ) ) ;
#120580=CARTESIAN_POINT ( 'NONE',  ( -6.700000000000016165, 12.50000000000000000, 4.330127018922196314 ) ) ;
#120581=VERTEX_POINT ( 'NONE', #109193 ) ;
#120582=FACE_OUTER_BOUND ( 'NONE', #29909, .T. ) ;
#120583=ADVANCED_FACE ( 'NONE', ( #40493 ), #87407, .T. ) ;
#120584=DIRECTION ( 'NONE',  ( 0.000000000000000000, 0.000000000000000000, -1.000000000000000000 ) ) ;
#120585=DIRECTION ( 'NONE',  ( 0.000000000000000000, 0.000000000000000000, 1.000000000000000000 ) ) ;
#120587=CARTESIAN_POINT ( 'NONE',  ( 15.59999999999988951, 2.500000000000000000, -0.3464101615137783474 ) ) ;
#120588=DIRECTION ( 'NONE',  ( 0.000000000000000000, 1.000000000000000000, 0.000000000000000000 ) ) ;
#120589=CARTESIAN_POINT ( 'NONE',  ( 14.34999999999989306, 12.50000000000000000, -2.511473670974877948 ) ) ;
#120590=CIRCLE ( 'NONE', #91343, 0.06509327318403745899 ) ;
#120591=EDGE_LOOP ( 'NONE', ( #48122, #76583, #76547, #39174 ) ) ;
#120592=VERTEX_POINT ( 'NONE', #79120 ) ;
#120593=CARTESIAN_POINT ( 'NONE',  ( -1.050000000000037348, 2.500000000000000000, -6.741600689897078169 ) ) ;
#120594=ORIENTED_EDGE ( 'NONE', *, *, #76930, .F. ) ;
#120595=DIRECTION ( 'NONE',  ( -4.274815082592931898E-19, -0.9999939076577903929, -0.003490651415223739937 ) ) ;
#120596=DIRECTION ( 'NONE',  ( 0.000000000000000000, 0.000000000000000000, 1.000000000000000000 ) ) ;
#120597=ADVANCED_FACE ( 'NONE', ( #88254 ), #58200, .T. ) ;
#120598=PLANE ( 'NONE',  #95003 ) ;
#120599=ORIENTED_EDGE ( 'NONE', *, *, #34689, .F. ) ;
#120600=EDGE_LOOP ( 'NONE', ( #94614, #86150, #41466, #81746 ) ) ;
#120601=FACE_BOUND ( 'NONE', #12855, .T. ) ;
#120602=ORIENTED_EDGE ( 'NONE', *, *, #37642, .T. ) ;
#120603=EDGE_CURVE ( 'NONE', #117308, #89205, #30019, .T. ) ;
#120604=DIRECTION ( 'NONE',  ( 0.000000000000000000, 0.000000000000000000, -1.000000000000000000 ) ) ;
#120606=CARTESIAN_POINT ( 'NONE',  ( -3.750000000000027978, 2.500000000000000000, 7.088010851410848190 ) ) ;
#120607=CARTESIAN_POINT ( 'NONE',  ( 2.949999999999943334, 2.500000000000000000, 6.395190528383296602 ) ) ;
#120608=AXIS2_PLACEMENT_3D ( 'NONE', #97436, #117062, #37877 ) ;
#120609=FACE_OUTER_BOUND ( 'NONE', #102643, .T. ) ;
#120610=CIRCLE ( 'NONE', #89304, 0.06509327318403745899 ) ;
#120611=CARTESIAN_POINT ( 'NONE',  ( 10.84999999999990905, 2.500000000000000000, -5.802370205355749988 ) ) ;
#120612=CARTESIAN_POINT ( 'NONE',  ( 0.1999999999999571565, 12.50000000000000000, 3.918623584224382839 ) ) ;
#120613=DIRECTION ( 'NONE',  ( -4.274815082592931898E-19, -0.9999939076577903929, -0.003490651415223739937 ) ) ;
#120614=EDGE_CURVE ( 'NONE', #56986, #47494, #38562, .T. ) ;
#120615=FACE_OUTER_BOUND ( 'NONE', #125912, .T. ) ;
#120616=CARTESIAN_POINT ( 'NONE',  ( -1.850000000000033840, 2.500000000000000000, 2.511473670974873507 ) ) ;
#120617=AXIS2_PLACEMENT_3D ( 'NONE', #67371, #56292, #15721 ) ;
#120618=EDGE_LOOP ( 'NONE', ( #32749, #81157, #116862, #57337 ) ) ;
#120619=VERTEX_POINT ( 'NONE', #49664 ) ;
#120620=ORIENTED_EDGE ( 'NONE', *, *, #11416, .F. ) ;
#120621=ORIENTED_EDGE ( 'NONE', *, *, #61669, .F. ) ;
#120622=CARTESIAN_POINT ( 'NONE',  ( -8.350000000000008527, 2.500000000000000000, 7.188010851410848723 ) ) ;
#120624=ORIENTED_EDGE ( 'NONE', *, *, #39990, .T. ) ;
#120625=ORIENTED_EDGE ( 'NONE', *, *, #94725, .T. ) ;
#120627=CARTESIAN_POINT ( 'NONE',  ( -6.050000000000020250, 12.50000000000000000, -6.841600689897078702 ) ) ;
#120628=AXIS2_PLACEMENT_3D ( 'NONE', #110999, #71752, #12800 ) ;
#120629=AXIS2_PLACEMENT_3D ( 'NONE', #117813, #28168, #36710 ) ;
#120630=VECTOR ( 'NONE', #93870, 1000.000000000000000 ) ;
#120631=CARTESIAN_POINT ( 'NONE',  ( 6.649999999999930189, 12.50000000000000000, -1.472243186433550122 ) ) ;
#120632=CARTESIAN_POINT ( 'NONE',  ( 12.69999999999990337, 12.50000000000000000, -4.676537180435978769 ) ) ;
#120633=FACE_OUTER_BOUND ( 'NONE', #74380, .T. ) ;
#120635=DIRECTION ( 'NONE',  ( 0.000000000000000000, 0.000000000000000000, -1.000000000000000000 ) ) ;
#120636=EDGE_LOOP ( 'NONE', ( #73437, #105957 ) ) ;
#120637=LINE ( 'NONE', #70898, #122847 ) ;
#120638=VERTEX_POINT ( 'NONE', #19533 ) ;
#120639=ADVANCED_FACE ( 'NONE', ( #69265 ), #104245, .T. ) ;
#120640=VERTEX_POINT ( 'NONE', #59499 ) ;
#120641=VERTEX_POINT ( 'NONE', #107270 ) ;
#120642=CARTESIAN_POINT ( 'NONE',  ( 3.949999999999938005, 2.500000000000000000, 6.741600689897071952 ) ) ;
#120643=ORIENTED_EDGE ( 'NONE', *, *, #93037, .F. ) ;
#120644=ADVANCED_FACE ( 'NONE', ( #17589 ), #49019, .T. ) ;
#120645=EDGE_LOOP ( 'NONE', ( #19712, #128825, #61764, #44888 ) ) ;
#120646=EDGE_LOOP ( 'NONE', ( #108341, #98124 ) ) ;
#120647=CONICAL_SURFACE ( 'NONE', #99728, 0.1000000000000002554, 0.003490658503988666988 ) ;
#120648=EDGE_CURVE ( 'NONE', #89168, #85675, #81261, .T. ) ;
#120649=CARTESIAN_POINT ( 'NONE',  ( 13.09999999999989839, 2.500000000000000000, -0.3464101615137783474 ) ) ;
#120650=FACE_OUTER_BOUND ( 'NONE', #35418, .T. ) ;
#120651=CARTESIAN_POINT ( 'NONE',  ( -8.150000000000009237, 12.50000000000000000, 6.148780366869520009 ) ) ;
#120652=CIRCLE ( 'NONE', #9830, 0.06509327318403745899 ) ;
#120653=LINE ( 'NONE', #99735, #52607 ) ;
#120654=CARTESIAN_POINT ( 'NONE',  ( -7.700000000000016165, 12.50000000000000000, 0.3464101615137735735 ) ) ;
#120655=EDGE_CURVE ( 'NONE', #97694, #72972, #95838, .T. ) ;
#120656=DIRECTION ( 'NONE',  ( -0.000000000000000000, -1.000000000000000000, -0.000000000000000000 ) ) ;
#120657=ADVANCED_FACE ( 'NONE', ( #28075 ), #58823, .T. ) ;
#120658=EDGE_CURVE ( 'NONE', #113211, #100972, #118906, .T. ) ;
#120659=AXIS2_PLACEMENT_3D ( 'NONE', #40277, #120765, #61201 ) ;
#120660=DIRECTION ( 'NONE',  ( -4.274815082592931898E-19, -0.9999939076577903929, -0.003490651415223739937 ) ) ;
#120661=ORIENTED_EDGE ( 'NONE', *, *, #120026, .F. ) ;
#120662=AXIS2_PLACEMENT_3D ( 'NONE', #63560, #55009, #53729 ) ;
#120663=DIRECTION ( 'NONE',  ( 0.000000000000000000, 0.000000000000000000, 1.000000000000000000 ) ) ;
#120664=EDGE_CURVE ( 'NONE', #84079, #125412, #125177, .T. ) ;
#120665=ORIENTED_EDGE ( 'NONE', *, *, #114199, .T. ) ;
#120667=LINE ( 'NONE', #91852, #71210 ) ;
#120668=ORIENTED_EDGE ( 'NONE', *, *, #95094, .F. ) ;
#120669=FACE_OUTER_BOUND ( 'NONE', #33547, .T. ) ;
#120670=CIRCLE ( 'NONE', #74691, 0.09999999999999982514 ) ;
#120671=EDGE_CURVE ( 'NONE', #125152, #97372, #111794, .T. ) ;
#120672=CARTESIAN_POINT ( 'NONE',  ( 9.999999999999948486, 2.500000000000000000, 4.230127018922196669 ) ) ;
#120673=VERTEX_POINT ( 'NONE', #61416 ) ;
#120674=ADVANCED_FACE ( 'NONE', ( #62697 ), #82984, .T. ) ;
#120675=AXIS2_PLACEMENT_3D ( 'NONE', #47407, #120010, #69609 ) ;
#120676=CONICAL_SURFACE ( 'NONE', #37058, 0.1000000000000000472, 0.003490658503988666988 ) ;
#120677=DIRECTION ( 'NONE',  ( -0.000000000000000000, -1.000000000000000000, -0.000000000000000000 ) ) ;
#120678=ORIENTED_EDGE ( 'NONE', *, *, #56586, .F. ) ;
#120679=ORIENTED_EDGE ( 'NONE', *, *, #50626, .F. ) ;
#120680=LINE ( 'NONE', #112795, #70636 ) ;
#120681=CARTESIAN_POINT ( 'NONE',  ( 2.499999999999983569, 2.500000000000000000, -0.1000000000000022815 ) ) ;
#120683=DIRECTION ( 'NONE',  ( 0.000000000000000000, 0.000000000000000000, -1.000000000000000000 ) ) ;
#120685=ORIENTED_EDGE ( 'NONE', *, *, #29487, .T. ) ;
#120686=DIRECTION ( 'NONE',  ( -0.000000000000000000, -1.000000000000000000, -0.000000000000000000 ) ) ;
#120687=VECTOR ( 'NONE', #54908, 1000.000000000000000 ) ;
#120688=ORIENTED_EDGE ( 'NONE', *, *, #33172, .F. ) ;
#120689=FACE_OUTER_BOUND ( 'NONE', #41956, .T. ) ;
#120690=CARTESIAN_POINT ( 'NONE',  ( -13.94999999999998863, 2.500000000000000000, 2.411473670974877415 ) ) ;
#120692=DIRECTION ( 'NONE',  ( -0.000000000000000000, -1.000000000000000000, -0.000000000000000000 ) ) ;
#120693=DIRECTION ( 'NONE',  ( 0.000000000000000000, 1.000000000000000000, 0.000000000000000000 ) ) ;
#120694=DIRECTION ( 'NONE',  ( -0.000000000000000000, 1.000000000000000000, -0.000000000000000000 ) ) ;
#120695=CARTESIAN_POINT ( 'NONE',  ( 4.799999999999937650, 12.50000000000000000, -3.983716857408426293 ) ) ;
#120696=ORIENTED_EDGE ( 'NONE', *, *, #106619, .F. ) ;
#120697=CIRCLE ( 'NONE', #99870, 0.1000000000000002554 ) ;
#120698=CARTESIAN_POINT ( 'NONE',  ( -6.050000000000018474, 12.50000000000000000, 2.511473670974873507 ) ) ;
#120699=ADVANCED_FACE ( 'NONE', ( #92803 ), #32615, .T. ) ;
#120700=CIRCLE ( 'NONE', #116480, 0.06509327318403745899 ) ;
#120701=DIRECTION ( 'NONE',  ( -0.000000000000000000, -1.000000000000000000, -0.000000000000000000 ) ) ;
#120702=DIRECTION ( 'NONE',  ( -0.000000000000000000, -1.000000000000000000, -0.000000000000000000 ) ) ;
#120703=EDGE_LOOP ( 'NONE', ( #55081, #62532 ) ) ;
#120704=AXIS2_PLACEMENT_3D ( 'NONE', #99307, #120235, #29282 ) ;
#120705=CIRCLE ( 'NONE', #1565, 0.06509327318403745899 ) ;
#120706=CARTESIAN_POINT ( 'NONE',  ( -3.350000000000028511, 2.500000000000000000, -2.757883832488654097 ) ) ;
#120707=ADVANCED_FACE ( 'NONE', ( #31314 ), #11649, .T. ) ;
#120708=AXIS2_PLACEMENT_3D ( 'NONE', #21139, #112112, #22458 ) ;
#120709=ORIENTED_EDGE ( 'NONE', *, *, #26816, .T. ) ;
#120711=DIRECTION ( 'NONE',  ( -4.274815082592931898E-19, -0.9999939076577903929, -0.003490651415223739937 ) ) ;
#120712=ORIENTED_EDGE ( 'NONE', *, *, #98439, .T. ) ;
#120713=CARTESIAN_POINT ( 'NONE',  ( 19.72570408286242127, -0.6078483229330700066, -4.299616118079172544 ) ) ;
#120714=DIRECTION ( 'NONE',  ( 0.000000000000000000, 0.000000000000000000, 1.000000000000000000 ) ) ;
#120715=CARTESIAN_POINT ( 'NONE',  ( 4.599999999999936584, 2.500000000000000000, 4.230127018922196669 ) ) ;
#120716=CIRCLE ( 'NONE', #62152, 0.06509327318403745899 ) ;
#120717=VERTEX_POINT ( 'NONE', #70568 ) ;
#120718=CARTESIAN_POINT ( 'NONE',  ( -11.64999999999999858, 12.50000000000000000, -5.802370205355746435 ) ) ;
#120719=FACE_OUTER_BOUND ( 'NONE', #82645, .T. ) ;
#120720=CARTESIAN_POINT ( 'NONE',  ( -2.500000000000030642, 2.500000000000000000, -5.022947341949754119 ) ) ;
#120721=ORIENTED_EDGE ( 'NONE', *, *, #82506, .F. ) ;
#120722=AXIS2_PLACEMENT_3D ( 'NONE', #106279, #56524, #103714 ) ;
#120723=ORIENTED_EDGE ( 'NONE', *, *, #90340, .T. ) ;
#120724=ORIENTED_EDGE ( 'NONE', *, *, #68252, .F. ) ;
#120725=CARTESIAN_POINT ( 'NONE',  ( -3.550000000000028688, 2.500000000000000000, 6.741600689897071952 ) ) ;
#120726=DIRECTION ( 'NONE',  ( 0.000000000000000000, 0.000000000000000000, 1.000000000000000000 ) ) ;
#120727=CARTESIAN_POINT ( 'NONE',  ( -5.650000000000019895, 2.500000000000000000, 2.411473670974873862 ) ) ;
#120728=FACE_BOUND ( 'NONE', #68808, .T. ) ;
#120729=ORIENTED_EDGE ( 'NONE', *, *, #94241, .F. ) ;
#120730=AXIS2_PLACEMENT_3D ( 'NONE', #5173, #34675, #66673 ) ;
#120731=DIRECTION ( 'NONE',  ( 0.000000000000000000, 1.000000000000000000, 0.000000000000000000 ) ) ;
#120732=CARTESIAN_POINT ( 'NONE',  ( 11.24999999999990763, 2.500000000000000000, -7.088010851410853519 ) ) ;
#120733=EDGE_LOOP ( 'NONE', ( #111423, #69163 ) ) ;
#120734=FACE_OUTER_BOUND ( 'NONE', #37579, .T. ) ;
#120735=EDGE_CURVE ( 'NONE', #18179, #30237, #26877, .T. ) ;
#120736=DIRECTION ( 'NONE',  ( 0.000000000000000000, 0.000000000000000000, 1.000000000000000000 ) ) ;
#120737=CIRCLE ( 'NONE', #22476, 0.06509327318403745899 ) ;
#120738=FACE_OUTER_BOUND ( 'NONE', #110005, .T. ) ;
#120739=CARTESIAN_POINT ( 'NONE',  ( -4.350000000000023626, 12.50000000000000000, 2.511473670974873507 ) ) ;
#120740=DIRECTION ( 'NONE',  ( 0.000000000000000000, 0.000000000000000000, 1.000000000000000000 ) ) ;
#120741=DIRECTION ( 'NONE',  ( -0.000000000000000000, 1.000000000000000000, -0.000000000000000000 ) ) ;
#120742=AXIS2_PLACEMENT_3D ( 'NONE', #40121, #119968, #38864 ) ;
#120743=CARTESIAN_POINT ( 'NONE',  ( 6.249999999999967137, 2.500000000000000000, -2.265063509461101798 ) ) ;
#120744=CIRCLE ( 'NONE', #118686, 0.06509327318403745899 ) ;
#120745=EDGE_CURVE ( 'NONE', #52849, #41301, #37355, .T. ) ;
#120746=VECTOR ( 'NONE', #111190, 1000.000000000000000 ) ;
#120747=ORIENTED_EDGE ( 'NONE', *, *, #120201, .F. ) ;
#120748=ORIENTED_EDGE ( 'NONE', *, *, #11123, .T. ) ;
#120749=VERTEX_POINT ( 'NONE', #3127 ) ;
#120750=ORIENTED_EDGE ( 'NONE', *, *, #38028, .T. ) ;
#120751=DIRECTION ( 'NONE',  ( 0.000000000000000000, 0.000000000000000000, 1.000000000000000000 ) ) ;
#120752=EDGE_CURVE ( 'NONE', #123701, #119499, #45758, .T. ) ;
#120753=CARTESIAN_POINT ( 'NONE',  ( -11.64999999999999680, 2.500000000000000000, -2.857883832488649745 ) ) ;
#120754=AXIS2_PLACEMENT_3D ( 'NONE', #63970, #35796, #65237 ) ;
#120755=ORIENTED_EDGE ( 'NONE', *, *, #112377, .T. ) ;
#120756=FACE_BOUND ( 'NONE', #104869, .T. ) ;
#120757=EDGE_CURVE ( 'NONE', #38170, #26678, #123027, .T. ) ;
#120758=CARTESIAN_POINT ( 'NONE',  ( -2.900000000000029665, 12.50000000000000000, 3.637306695894644726 ) ) ;
#120760=AXIS2_PLACEMENT_3D ( 'NONE', #31010, #93134, #122588 ) ;
#120761=VECTOR ( 'NONE', #38368, 1000.000000000000000 ) ;
#120762=EDGE_CURVE ( 'NONE', #113663, #60541, #77054, .T. ) ;
#120763=FACE_OUTER_BOUND ( 'NONE', #5959, .T. ) ;
#120764=CARTESIAN_POINT ( 'NONE',  ( -8.750000000000010658, 12.50000000000000000, -1.472243186433550122 ) ) ;
#120765=DIRECTION ( 'NONE',  ( 0.000000000000000000, 1.000000000000000000, 0.000000000000000000 ) ) ;
#120766=CARTESIAN_POINT ( 'NONE',  ( 6.249999999999934275, 2.500000000000000000, -7.088010851410853519 ) ) ;
#120767=DIRECTION ( 'NONE',  ( 0.000000000000000000, 0.000000000000000000, 1.000000000000000000 ) ) ;
#120768=ADVANCED_FACE ( 'NONE', ( #12911 ), #73154, .T. ) ;
#120769=DIRECTION ( 'NONE',  ( -0.000000000000000000, 1.000000000000000000, -0.000000000000000000 ) ) ;
#120771=ORIENTED_EDGE ( 'NONE', *, *, #78094, .T. ) ;
#120772=ORIENTED_EDGE ( 'NONE', *, *, #19716, .F. ) ;
#120773=ORIENTED_EDGE ( 'NONE', *, *, #118769, .F. ) ;
#120774=ORIENTED_EDGE ( 'NONE', *, *, #28739, .T. ) ;
#120775=ORIENTED_EDGE ( 'NONE', *, *, #58112, .F. ) ;
#120777=EDGE_LOOP ( 'NONE', ( #89124, #86881 ) ) ;
#120778=DIRECTION ( 'NONE',  ( -0.000000000000000000, 1.000000000000000000, -0.000000000000000000 ) ) ;
#120779=CARTESIAN_POINT ( 'NONE',  ( 16.31212829106973672, -2.500000000000129674, 6.358241997069454143 ) ) ;
#120780=LINE ( 'NONE', #31138, #129461 ) ;
#120781=DIRECTION ( 'NONE',  ( 0.000000000000000000, 0.000000000000000000, 1.000000000000000000 ) ) ;
#120782=VERTEX_POINT ( 'NONE', #101330 ) ;
#120783=CARTESIAN_POINT ( 'NONE',  ( -10.40000000000000213, 2.500000000000000000, 0.6928203230275494784 ) ) ;
#120784=AXIS2_PLACEMENT_3D ( 'NONE', #121282, #60456, #100362 ) ;
#120785=ORIENTED_EDGE ( 'NONE', *, *, #79974, .F. ) ;
#120786=EDGE_CURVE ( 'NONE', #118189, #95937, #64519, .T. ) ;
#120787=CIRCLE ( 'NONE', #49797, 0.06509327318403745899 ) ;
#120788=ORIENTED_EDGE ( 'NONE', *, *, #49179, .T. ) ;
#120789=CARTESIAN_POINT ( 'NONE',  ( 4.199999999999941558, 12.50000000000000000, -4.395220292106239768 ) ) ;
#120790=LINE ( 'NONE', #70408, #57339 ) ;
#120791=FACE_OUTER_BOUND ( 'NONE', #48246, .T. ) ;
#120792=EDGE_CURVE ( 'NONE', #72819, #119417, #14333, .T. ) ;
#120793=ORIENTED_EDGE ( 'NONE', *, *, #87357, .F. ) ;
#120794=CIRCLE ( 'NONE', #104078, 0.06509327318403745899 ) ;
#120797=DIRECTION ( 'NONE',  ( -0.000000000000000000, -1.000000000000000000, -0.000000000000000000 ) ) ;
#120798=VECTOR ( 'NONE', #118534, 1000.000000000000000 ) ;
#120799=AXIS2_PLACEMENT_3D ( 'NONE', #21793, #71513, #110160 ) ;
#120800=CARTESIAN_POINT ( 'NONE',  ( 8.299999999999922551, 2.500000000000000000, -2.385244779468109755E-15 ) ) ;
#120801=DIRECTION ( 'NONE',  ( 0.000000000000000000, 0.000000000000000000, -1.000000000000000000 ) ) ;
#120802=DIRECTION ( 'NONE',  ( 0.000000000000000000, 1.000000000000000000, 0.000000000000000000 ) ) ;
#120803=VERTEX_POINT ( 'NONE', #30670 ) ;
#120804=ADVANCED_FACE ( 'NONE', ( #52229 ), #66574, .T. ) ;
#120805=CARTESIAN_POINT ( 'NONE',  ( -6.850000000000017408, 2.500000000000000000, -6.741600689897077281 ) ) ;
#120806=EDGE_CURVE ( 'NONE', #124753, #118132, #87496, .T. ) ;
#120807=EDGE_CURVE ( 'NONE', #59372, #43527, #72518, .T. ) ;
#120808=ORIENTED_EDGE ( 'NONE', *, *, #65474, .T. ) ;
#120809=CARTESIAN_POINT ( 'NONE',  ( 10.06913504599025977, -2.500000000000000444, 8.158951466667735630 ) ) ;
#120810=CIRCLE ( 'NONE', #125013, 0.06509327318403745899 ) ;
#120811=ORIENTED_EDGE ( 'NONE', *, *, #98229, .F. ) ;
#120812=CARTESIAN_POINT ( 'NONE',  ( -5.600000000000023626, 12.50000000000000000, -4.048810130592463530 ) ) ;
#120813=EDGE_CURVE ( 'NONE', #93332, #26619, #10155, .T. ) ;
#120814=DIRECTION ( 'NONE',  ( 0.000000000000000000, 1.000000000000000000, 0.000000000000000000 ) ) ;
#120815=CARTESIAN_POINT ( 'NONE',  ( -3.350000000000031619, 12.50000000000000000, -5.802370205355749988 ) ) ;
#120816=CONICAL_SURFACE ( 'NONE', #51867, 0.09999999999999982514, 0.003490658503988666988 ) ;
#120817=CARTESIAN_POINT ( 'NONE',  ( -11.24999999999999822, 2.500000000000000000, 5.802370205355744659 ) ) ;
#120818=EDGE_LOOP ( 'NONE', ( #50585, #89095, #29216, #22766 ) ) ;
#120819=ADVANCED_FACE ( 'NONE', ( #125466 ), #41567, .T. ) ;
#120820=DIRECTION ( 'NONE',  ( 0.000000000000000000, 0.000000000000000000, -1.000000000000000000 ) ) ;
#120821=AXIS2_PLACEMENT_3D ( 'NONE', #5756, #27332, #56785 ) ;
#120822=EDGE_CURVE ( 'NONE', #38829, #42322, #116750, .T. ) ;
#120823=MECHANICAL_DESIGN_GEOMETRIC_PRESENTATION_REPRESENTATION('',(#47672),#7945);
#120824=CARTESIAN_POINT ( 'NONE',  ( 0.6499999999999561684, 2.500000000000000000, 1.818653347947321475 ) ) ;
#120825=ORIENTED_EDGE ( 'NONE', *, *, #96267, .T. ) ;
#120826=ORIENTED_EDGE ( 'NONE', *, *, #53008, .F. ) ;
#120827=ORIENTED_EDGE ( 'NONE', *, *, #72040, .F. ) ;
#120828=CARTESIAN_POINT ( 'NONE',  ( -10.60000000000000320, 12.50000000000000000, -4.676537180435973440 ) ) ;
#120829=CARTESIAN_POINT ( 'NONE',  ( -1.050000000000037348, 2.500000000000000000, -2.411473670974877859 ) ) ;
#120830=CARTESIAN_POINT ( 'NONE',  ( -1.250000000000036193, 2.500000000000000000, 1.572243186433545548 ) ) ;
#120831=DIRECTION ( 'NONE',  ( 0.000000000000000000, -0.9999939076577903929, 0.003490651415223739937 ) ) ;
#120832=VECTOR ( 'NONE', #126595, 1000.000000000000000 ) ;
#120833=CARTESIAN_POINT ( 'NONE',  ( -11.24999999999999822, 12.50000000000000000, 5.802370205355744659 ) ) ;
#120834=CIRCLE ( 'NONE', #35168, 0.06509327318403745899 ) ;
#120835=DIRECTION ( 'NONE',  ( 0.000000000000000000, 0.000000000000000000, 1.000000000000000000 ) ) ;
#120836=CIRCLE ( 'NONE', #33025, 0.1000000000000000472 ) ;
#120837=DIRECTION ( 'NONE',  ( -0.000000000000000000, 1.000000000000000000, -0.000000000000000000 ) ) ;
#120838=DIRECTION ( 'NONE',  ( 0.000000000000000000, -0.9999939076577903929, 0.003490651415223739937 ) ) ;
#120839=LINE ( 'NONE', #97966, #102774 ) ;
#120840=CONICAL_SURFACE ( 'NONE', #43210, 0.1000000000000000472, 0.003490658503988666988 ) ;
#120841=ORIENTED_EDGE ( 'NONE', *, *, #121130, .F. ) ;
#120843=CIRCLE ( 'NONE', #74880, 0.06509327318403745899 ) ;
#120844=FACE_OUTER_BOUND ( 'NONE', #9552, .T. ) ;
#120845=DIRECTION ( 'NONE',  ( 0.000000000000000000, 0.000000000000000000, 1.000000000000000000 ) ) ;
#120846=DIRECTION ( 'NONE',  ( -0.000000000000000000, 1.000000000000000000, -0.000000000000000000 ) ) ;
#120847=ORIENTED_EDGE ( 'NONE', *, *, #126434, .F. ) ;
#120848=CARTESIAN_POINT ( 'NONE',  ( -12.09999999999999609, 2.500000000000000000, -0.5928203230275500557 ) ) ;
#120850=CIRCLE ( 'NONE', #114574, 0.06509327318403745899 ) ;
#120851=EDGE_CURVE ( 'NONE', #98415, #23253, #60347, .T. ) ;
#120853=FACE_OUTER_BOUND ( 'NONE', #13090, .T. ) ;
#120855=ORIENTED_EDGE ( 'NONE', *, *, #93055, .F. ) ;
#120856=DIRECTION ( 'NONE',  ( 0.000000000000000000, -0.9999939076577903929, 0.003490651415223739937 ) ) ;
#120857=EDGE_CURVE ( 'NONE', #79541, #2654, #110500, .T. ) ;
#120858=EDGE_LOOP ( 'NONE', ( #65288, #27713 ) ) ;
#120859=ORIENTED_EDGE ( 'NONE', *, *, #79877, .T. ) ;
#120860=DIRECTION ( 'NONE',  ( -0.000000000000000000, -1.000000000000000000, -0.000000000000000000 ) ) ;
#120861=DIRECTION ( 'NONE',  ( 0.000000000000000000, 0.000000000000000000, -1.000000000000000000 ) ) ;
#120862=CARTESIAN_POINT ( 'NONE',  ( 8.749999999999923617, 2.500000000000000000, 1.372243186433545370 ) ) ;
#120863=CARTESIAN_POINT ( 'NONE',  ( 9.399999999999915090, 2.500000000000000000, 3.983716857408420964 ) ) ;
#120864=ORIENTED_EDGE ( 'NONE', *, *, #111186, .F. ) ;
#120865=CIRCLE ( 'NONE', #106208, 0.1000000000000002554 ) ;
#120866=CIRCLE ( 'NONE', #28948, 0.1000000000000002554 ) ;
#120868=EDGE_LOOP ( 'NONE', ( #30925, #86728, #65604, #87259 ) ) ;
#120869=VECTOR ( 'NONE', #101937, 1000.000000000000000 ) ;
#120870=DIRECTION ( 'NONE',  ( 0.000000000000000000, 0.000000000000000000, -1.000000000000000000 ) ) ;
#120871=CARTESIAN_POINT ( 'NONE',  ( -2.100000000000034284, 12.50000000000000000, -2.385244779468109755E-15 ) ) ;
#120872=VERTEX_POINT ( 'NONE', #44324 ) ;
#120873=AXIS2_PLACEMENT_3D ( 'NONE', #129041, #117230, #47243 ) ;
#120874=CONICAL_SURFACE ( 'NONE', #58209, 0.09999999999999982514, 0.003490658503988666988 ) ;
#120875=ORIENTED_EDGE ( 'NONE', *, *, #53036, .F. ) ;
#120876=ORIENTED_EDGE ( 'NONE', *, *, #79429, .F. ) ;
#120877=ORIENTED_EDGE ( 'NONE', *, *, #121081, .T. ) ;
#120878=DIRECTION ( 'NONE',  ( -0.000000000000000000, 1.000000000000000000, -0.000000000000000000 ) ) ;
#120879=CARTESIAN_POINT ( 'NONE',  ( 8.512291507278087366, 1.500000000000128120, 9.502944100741384403 ) ) ;
#120880=DIRECTION ( 'NONE',  ( -0.000000000000000000, -1.000000000000000000, -0.000000000000000000 ) ) ;
#120881=FACE_BOUND ( 'NONE', #124725, .T. ) ;
#120882=CARTESIAN_POINT ( 'NONE',  ( -3.749999999999991118, 2.500000000000000000, 2.265063509461097357 ) ) ;
#120885=CARTESIAN_POINT ( 'NONE',  ( -0.6500000000000403233, 12.50000000000000000, 1.818653347947321475 ) ) ;
#120886=DIRECTION ( 'NONE',  ( -0.000000000000000000, 1.000000000000000000, -0.000000000000000000 ) ) ;
#120887=CARTESIAN_POINT ( 'NONE',  ( -0.4000000000000392131, 12.50000000000000000, -5.088040615133791356 ) ) ;
#120888=CARTESIAN_POINT ( 'NONE',  ( 12.49999999999993605, 12.50000000000000000, 0.06509327318403515528 ) ) ;
#120889=CARTESIAN_POINT ( 'NONE',  ( -8.750000000000010658, 2.500000000000000000, -7.088010851410848190 ) ) ;
#120890=CIRCLE ( 'NONE', #116686, 0.09999999999999982514 ) ;
#120891=EDGE_CURVE ( 'NONE', #88147, #123047, #74444, .T. ) ;
#120892=DIRECTION ( 'NONE',  ( -0.000000000000000000, 1.000000000000000000, -0.000000000000000000 ) ) ;
#120893=VERTEX_POINT ( 'NONE', #115636 ) ;
#120894=ORIENTED_EDGE ( 'NONE', *, *, #29899, .T. ) ;
#120895=ORIENTED_EDGE ( 'NONE', *, *, #113676, .T. ) ;
#120896=ORIENTED_EDGE ( 'NONE', *, *, #86348, .F. ) ;
#120897=VERTEX_POINT ( 'NONE', #56702 ) ;
#120898=AXIS2_PLACEMENT_3D ( 'NONE', #123879, #74803, #95733 ) ;
#120899=DIRECTION ( 'NONE',  ( 0.000000000000000000, 0.000000000000000000, -1.000000000000000000 ) ) ;
#120900=EDGE_CURVE ( 'NONE', #79354, #63146, #65242, .T. ) ;
#120901=DIRECTION ( 'NONE',  ( -4.274815082592931898E-19, -0.9999939076577903929, -0.003490651415223739937 ) ) ;
#120902=VERTEX_POINT ( 'NONE', #25993 ) ;
#120903=FACE_BOUND ( 'NONE', #92839, .T. ) ;
#120904=ADVANCED_FACE ( 'NONE', ( #16133 ), #124184, .T. ) ;
#120905=LINE ( 'NONE', #81622, #127211 ) ;
#120906=VECTOR ( 'NONE', #50979, 1000.000000000000000 ) ;
#120908=EDGE_CURVE ( 'NONE', #81253, #46586, #5037, .T. ) ;
#120909=EDGE_CURVE ( 'NONE', #64039, #31018, #74997, .T. ) ;
#120910=VERTEX_POINT ( 'NONE', #24056 ) ;
#120911=CARTESIAN_POINT ( 'NONE',  ( 6.899999999999926636, 2.500000000000000000, 0.3464101615137736845 ) ) ;
#120912=DIRECTION ( 'NONE',  ( 0.000000000000000000, -0.000000000000000000, 1.000000000000000000 ) ) ;
#120913=DIRECTION ( 'NONE',  ( 0.000000000000000000, 0.000000000000000000, -1.000000000000000000 ) ) ;
#120914=EDGE_CURVE ( 'NONE', #97281, #113533, #91719, .T. ) ;
#120915=CARTESIAN_POINT ( 'NONE',  ( -8.350000000000013856, 12.50000000000000000, -2.099970236277064473 ) ) ;
#120916=VERTEX_POINT ( 'NONE', #94080 ) ;
#120917=CIRCLE ( 'NONE', #125129, 0.06509327318403745899 ) ;
#120918=DIRECTION ( 'NONE',  ( -4.274815082592931898E-19, -0.9999939076577903929, -0.003490651415223739937 ) ) ;
#120919=CONICAL_SURFACE ( 'NONE', #5882, 0.1000000000000002554, 0.003490658503988666988 ) ;
#120920=ORIENTED_EDGE ( 'NONE', *, *, #105832, .F. ) ;
#120921=ORIENTED_EDGE ( 'NONE', *, *, #19271, .F. ) ;
#120922=DIRECTION ( 'NONE',  ( 0.000000000000000000, 1.000000000000000000, 0.000000000000000000 ) ) ;
#120923=DIRECTION ( 'NONE',  ( 0.000000000000000000, 0.000000000000000000, 1.000000000000000000 ) ) ;
#120924=EDGE_LOOP ( 'NONE', ( #108608, #90714 ) ) ;
#120925=CARTESIAN_POINT ( 'NONE',  ( -3.100000000000028955, 12.50000000000000000, 3.983716857408420964 ) ) ;
#120926=FACE_OUTER_BOUND ( 'NONE', #85761, .T. ) ;
#120927=CARTESIAN_POINT ( 'NONE',  ( -1.250000000000001554, 2.500000000000000000, 6.595190528383296780 ) ) ;
#120929=FACE_OUTER_BOUND ( 'NONE', #92811, .T. ) ;
#120930=EDGE_LOOP ( 'NONE', ( #62748, #46997 ) ) ;
#120931=DIRECTION ( 'NONE',  ( 0.000000000000000000, 0.000000000000000000, 1.000000000000000000 ) ) ;
#120932=EDGE_LOOP ( 'NONE', ( #91072, #111134, #72822, #97203 ) ) ;
#120933=DIRECTION ( 'NONE',  ( 0.000000000000000000, 0.000000000000000000, 1.000000000000000000 ) ) ;
#120934=AXIS2_PLACEMENT_3D ( 'NONE', #115650, #86843, #76394 ) ;
#120935=VECTOR ( 'NONE', #75775, 1000.000000000000000 ) ;
#120936=ORIENTED_EDGE ( 'NONE', *, *, #70280, .F. ) ;
#120937=DIRECTION ( 'NONE',  ( 0.000000000000000000, 0.000000000000000000, -1.000000000000000000 ) ) ;
#120938=ORIENTED_EDGE ( 'NONE', *, *, #50560, .F. ) ;
#120939=CARTESIAN_POINT ( 'NONE',  ( 12.89999999999990088, 2.500000000000000000, 4.230127018922196669 ) ) ;
#120940=DIRECTION ( 'NONE',  ( -0.000000000000000000, 1.000000000000000000, -0.000000000000000000 ) ) ;
#120941=DIRECTION ( 'NONE',  ( 0.000000000000000000, 0.000000000000000000, 1.000000000000000000 ) ) ;
#120942=CARTESIAN_POINT ( 'NONE',  ( 0.7999999999999553024, 2.500000000000000000, -4.330127018922201643 ) ) ;
#120943=CARTESIAN_POINT ( 'NONE',  ( 10.44999999999991047, 2.500000000000000000, -6.495190528383302464 ) ) ;
#120944=ORIENTED_EDGE ( 'NONE', *, *, #84271, .T. ) ;
#120945=ORIENTED_EDGE ( 'NONE', *, *, #54609, .T. ) ;
#120946=ORIENTED_EDGE ( 'NONE', *, *, #18417, .F. ) ;
#120947=CARTESIAN_POINT ( 'NONE',  ( -10.40000000000000391, 2.500000000000000000, -3.737306695894645259 ) ) ;
#120948=DIRECTION ( 'NONE',  ( 0.000000000000000000, -0.9999939076577903929, 0.003490651415223739937 ) ) ;
#120949=CARTESIAN_POINT ( 'NONE',  ( 5.649999999999934630, 12.50000000000000000, 6.213873640053559022 ) ) ;
#120950=EDGE_CURVE ( 'NONE', #7073, #78283, #34536, .T. ) ;
#120951=CONICAL_SURFACE ( 'NONE', #22681, 0.1000000000000000472, 0.003490658503988666988 ) ;
#120952=ORIENTED_EDGE ( 'NONE', *, *, #46214, .F. ) ;
#120953=EDGE_LOOP ( 'NONE', ( #58902, #22194, #57688, #102283 ) ) ;
#120954=VERTEX_POINT ( 'NONE', #14840 ) ;
#120955=EDGE_CURVE ( 'NONE', #41978, #115959, #39427, .T. ) ;
#120956=DIRECTION ( 'NONE',  ( 0.000000000000000000, 1.000000000000000000, 0.000000000000000000 ) ) ;
#120957=EDGE_CURVE ( 'NONE', #115043, #104608, #96012, .T. ) ;
#120958=ORIENTED_EDGE ( 'NONE', *, *, #53424, .F. ) ;
#120959=CARTESIAN_POINT ( 'NONE',  ( -4.293440603042597559E-14, 2.500000000000000000, 5.022947341949748790 ) ) ;
#120960=CARTESIAN_POINT ( 'NONE',  ( 11.64999999999990798, 2.500000000000000000, -2.757883832488654097 ) ) ;
#120962=CONICAL_SURFACE ( 'NONE', #79212, 0.1000000000000002554, 0.003490658503988666988 ) ;
#120963=CARTESIAN_POINT ( 'NONE',  ( -6.900000000000019007, 12.50000000000000000, -0.3464101615137783474 ) ) ;
#120964=DIRECTION ( 'NONE',  ( -0.000000000000000000, 1.000000000000000000, -0.000000000000000000 ) ) ;
#120965=AXIS2_PLACEMENT_3D ( 'NONE', #117713, #98094, #67313 ) ;
#120966=FACE_OUTER_BOUND ( 'NONE', #79420, .T. ) ;
#120967=EDGE_CURVE ( 'NONE', #41467, #69086, #114988, .T. ) ;
#120968=DIRECTION ( 'NONE',  ( 0.000000000000000000, 1.000000000000000000, 0.000000000000000000 ) ) ;
#120969=FACE_OUTER_BOUND ( 'NONE', #33377, .T. ) ;
#120970=EDGE_CURVE ( 'NONE', #43475, #62131, #121298, .T. ) ;
#120971=CARTESIAN_POINT ( 'NONE',  ( -6.650000000000014566, 12.50000000000000000, 1.472243186433545459 ) ) ;
#120972=CONICAL_SURFACE ( 'NONE', #95845, 0.1000000000000002554, 0.003490658503988666988 ) ;
#120973=EDGE_LOOP ( 'NONE', ( #117466, #31170, #4935, #66635 ) ) ;
#120974=AXIS2_PLACEMENT_3D ( 'NONE', #126288, #77182, #97465 ) ;
#120975=EDGE_CURVE ( 'NONE', #124470, #8336, #106472, .T. ) ;
#120976=CARTESIAN_POINT ( 'NONE',  ( 9.349999999999916156, 12.50000000000000000, 6.148780366869520009 ) ) ;
#120977=ADVANCED_FACE ( 'NONE', ( #35804 ), #69773, .T. ) ;
#120978=CIRCLE ( 'NONE', #64530, 0.06509327318403745899 ) ;
#120979=FACE_OUTER_BOUND ( 'NONE', #36178, .T. ) ;
#120980=ORIENTED_EDGE ( 'NONE', *, *, #87571, .F. ) ;
#120981=ORIENTED_EDGE ( 'NONE', *, *, #65311, .T. ) ;
#120983=DIRECTION ( 'NONE',  ( -0.000000000000000000, 1.000000000000000000, -0.000000000000000000 ) ) ;
#120984=DIRECTION ( 'NONE',  ( -0.000000000000000000, -1.000000000000000000, -0.000000000000000000 ) ) ;
#120985=ADVANCED_FACE ( 'NONE', ( #78966 ), #88092, .T. ) ;
#120986=AXIS2_PLACEMENT_3D ( 'NONE', #128647, #78892, #46847 ) ;
#120987=CARTESIAN_POINT ( 'NONE',  ( -9.550000000000002487, 2.500000000000000000, 6.495190528383297135 ) ) ;
#120988=CARTESIAN_POINT ( 'NONE',  ( -8.350000000000012079, 12.50000000000000000, -1.537336459617587581 ) ) ;
#120989=AXIS2_PLACEMENT_3D ( 'NONE', #3951, #110682, #60941 ) ;
#120990=FACE_OUTER_BOUND ( 'NONE', #111088, .T. ) ;
#120991=CARTESIAN_POINT ( 'NONE',  ( 9.599999999999914380, 2.500000000000000000, 3.537306695894645081 ) ) ;
#120992=CARTESIAN_POINT ( 'NONE',  ( 0.6499999999999543920, 12.50000000000000000, 6.906693963081109722 ) ) ;
#120993=CARTESIAN_POINT ( 'NONE',  ( 12.29999999999990656, 2.500000000000000000, 4.083716857408421497 ) ) ;
#120994=AXIS2_PLACEMENT_3D ( 'NONE', #109158, #10334, #20803 ) ;
#120995=ORIENTED_EDGE ( 'NONE', *, *, #2856, .T. ) ;
#120996=EDGE_LOOP ( 'NONE', ( #14526, #14355 ) ) ;
#120997=VERTEX_POINT ( 'NONE', #118873 ) ;
#120998=AXIS2_PLACEMENT_3D ( 'NONE', #125503, #94758, #46963 ) ;
#120999=ORIENTED_EDGE ( 'NONE', *, *, #122607, .F. ) ;
#121000=EDGE_LOOP ( 'NONE', ( #90532, #30304 ) ) ;
#121001=CARTESIAN_POINT ( 'NONE',  ( -3.950000000000026379, 12.50000000000000000, 6.841600689897072485 ) ) ;
#121002=DIRECTION ( 'NONE',  ( 0.000000000000000000, 1.000000000000000000, 0.000000000000000000 ) ) ;
#121003=VERTEX_POINT ( 'NONE', #128727 ) ;
#121005=DIRECTION ( 'NONE',  ( 0.000000000000000000, 0.000000000000000000, -1.000000000000000000 ) ) ;
#121006=CIRCLE ( 'NONE', #8126, 0.06509327318403745899 ) ;
#121007=DIRECTION ( 'NONE',  ( 0.000000000000000000, 0.000000000000000000, -1.000000000000000000 ) ) ;
#121008=CARTESIAN_POINT ( 'NONE',  ( 6.849999999999930367, 2.500000000000000000, -6.248780366869526759 ) ) ;
#121009=VERTEX_POINT ( 'NONE', #38403 ) ;
#121010=PLANE ( 'NONE',  #43265 ) ;
#121011=CIRCLE ( 'NONE', #58336, 0.09999999999999982514 ) ;
#121012=LINE ( 'NONE', #22834, #125172 ) ;
#121013=ORIENTED_EDGE ( 'NONE', *, *, #30229, .F. ) ;
#121014=CIRCLE ( 'NONE', #108488, 0.06509327318403745899 ) ;
#121015=ADVANCED_FACE ( 'NONE', ( #97299 ), #92041, .T. ) ;
#121016=ORIENTED_EDGE ( 'NONE', *, *, #75700, .T. ) ;
#121017=EDGE_LOOP ( 'NONE', ( #47908, #76026, #35767, #72120 ) ) ;
#121018=VERTEX_POINT ( 'NONE', #49509 ) ;
#121019=CARTESIAN_POINT ( 'NONE',  ( 3.349999999999945466, 2.500000000000000000, -7.188010851410854052 ) ) ;
#121021=CARTESIAN_POINT ( 'NONE',  ( 9.149999999999916866, 2.500000000000000000, 5.702370205355745014 ) ) ;
#121022=CARTESIAN_POINT ( 'NONE',  ( -8.350000000000013856, 2.500000000000000000, 2.265063509461097357 ) ) ;
#121023=ORIENTED_EDGE ( 'NONE', *, *, #35993, .F. ) ;
#121024=CONICAL_SURFACE ( 'NONE', #89634, 0.09999999999999982514, 0.003490658503988666988 ) ;
#121025=AXIS2_PLACEMENT_3D ( 'NONE', #122350, #22868, #64060 ) ;
#121026=DIRECTION ( 'NONE',  ( -0.000000000000000000, 1.000000000000000000, -0.000000000000000000 ) ) ;
#121027=VERTEX_POINT ( 'NONE', #107762 ) ;
#121028=LINE ( 'NONE', #40561, #99698 ) ;
#121029=CARTESIAN_POINT ( 'NONE',  ( 19.09982477502543219, -0.5559300837585612332, -4.454172625795868257 ) ) ;
#121030=CIRCLE ( 'NONE', #29109, 0.06509327318403745899 ) ;
#121031=DIRECTION ( 'NONE',  ( -0.000000000000000000, -1.000000000000000000, -0.000000000000000000 ) ) ;
#121032=CARTESIAN_POINT ( 'NONE',  ( -2.499999999999996003, 2.500000000000000000, -2.276824562219559311E-15 ) ) ;
#121033=ORIENTED_EDGE ( 'NONE', *, *, #110001, .T. ) ;
#121034=CONICAL_SURFACE ( 'NONE', #64594, 0.1000000000000002554, 0.003490658503988666988 ) ;
#121035=CIRCLE ( 'NONE', #75067, 0.1000000000000000472 ) ;
#121036=EDGE_LOOP ( 'NONE', ( #107760, #91894, #82491, #52550 ) ) ;
#121037=VERTEX_POINT ( 'NONE', #29852 ) ;
#121038=DIRECTION ( 'NONE',  ( -4.274815082592931898E-19, -0.9999939076577903929, -0.003490651415223739937 ) ) ;
#121039=CARTESIAN_POINT ( 'NONE',  ( 9.799999999999913669, 12.50000000000000000, 4.676537180435972552 ) ) ;
#121040=FACE_BOUND ( 'NONE', #37431, .T. ) ;
#121041=CARTESIAN_POINT ( 'NONE',  ( -13.74999999999998934, 2.500000000000000000, 2.757883832488653209 ) ) ;
#121042=CARTESIAN_POINT ( 'NONE',  ( -7.500000000000015099, 12.50000000000000000, -0.6928203230275541413 ) ) ;
#121043=CARTESIAN_POINT ( 'NONE',  ( -9.150000000000009237, 2.500000000000000000, -2.857883832488653741 ) ) ;
#121044=CIRCLE ( 'NONE', #18549, 0.09999999999999982514 ) ;
#121045=PLANE ( 'NONE',  #40097 ) ;
#121047=CARTESIAN_POINT ( 'NONE',  ( -10.40000000000000213, 12.50000000000000000, 5.088040615133786027 ) ) ;
#121049=DIRECTION ( 'NONE',  ( 0.000000000000000000, 1.000000000000000000, 0.000000000000000000 ) ) ;
#121050=AXIS2_PLACEMENT_3D ( 'NONE', #51973, #1559, #119393 ) ;
#121051=EDGE_CURVE ( 'NONE', #43024, #32323, #58672, .T. ) ;
#121052=CONICAL_SURFACE ( 'NONE', #18641, 0.1000000000000000472, 0.003490658503988666988 ) ;
#121053=DIRECTION ( 'NONE',  ( 0.000000000000000000, 0.000000000000000000, -1.000000000000000000 ) ) ;
#121054=ORIENTED_EDGE ( 'NONE', *, *, #98973, .F. ) ;
#121055=EDGE_LOOP ( 'NONE', ( #90561, #55276, #13054, #107249 ) ) ;
#121056=DIRECTION ( 'NONE',  ( 0.000000000000000000, 1.000000000000000000, 0.000000000000000000 ) ) ;
#121058=CARTESIAN_POINT ( 'NONE',  ( 5.849999999999933031, 2.500000000000000000, 7.088010851410848190 ) ) ;
#121059=FACE_BOUND ( 'NONE', #128040, .T. ) ;
#121060=EDGE_CURVE ( 'NONE', #86814, #73847, #77013, .T. ) ;
#121061=DIRECTION ( 'NONE',  ( 0.000000000000000000, 0.000000000000000000, 1.000000000000000000 ) ) ;
#121062=CIRCLE ( 'NONE', #75097, 0.06509327318403745899 ) ;
#121063=AXIS2_PLACEMENT_3D ( 'NONE', #54793, #34549, #83637 ) ;
#121064=CIRCLE ( 'NONE', #56300, 0.1000000000000002554 ) ;
#121065=CARTESIAN_POINT ( 'NONE',  ( 97.50000000000000000, 0.000000000000000000, 0.000000000000000000 ) ) ;
#121066=EDGE_CURVE ( 'NONE', #23803, #86766, #27288, .T. ) ;
#121067=EDGE_CURVE ( 'NONE', #87887, #11509, #20038, .T. ) ;
#121069=DIRECTION ( 'NONE',  ( 0.000000000000000000, 0.000000000000000000, 1.000000000000000000 ) ) ;
#121070=ADVANCED_FACE ( 'NONE', ( #87463 ), #18879, .T. ) ;
#121071=EDGE_CURVE ( 'NONE', #84610, #269, #69053, .T. ) ;
#121072=DIRECTION ( 'NONE',  ( 0.000000000000000000, 0.000000000000000000, -1.000000000000000000 ) ) ;
#121073=EDGE_CURVE ( 'NONE', #111655, #51736, #81578, .T. ) ;
#121074=CIRCLE ( 'NONE', #89680, 0.06509327318403741736 ) ;
#121075=VERTEX_POINT ( 'NONE', #27915 ) ;
#121076=DIRECTION ( 'NONE',  ( -4.274815082592931898E-19, -0.9999939076577903929, -0.003490651415223739937 ) ) ;
#121077=DIRECTION ( 'NONE',  ( 0.000000000000000000, 0.000000000000000000, -1.000000000000000000 ) ) ;
#121078=CIRCLE ( 'NONE', #98086, 0.06509327318403745899 ) ;
#121079=DIRECTION ( 'NONE',  ( 0.000000000000000000, 0.000000000000000000, 1.000000000000000000 ) ) ;
#121080=DIRECTION ( 'NONE',  ( -0.000000000000000000, -1.000000000000000000, -0.000000000000000000 ) ) ;
#121081=EDGE_CURVE ( 'NONE', #51026, #56576, #41888, .T. ) ;
#121082=EDGE_LOOP ( 'NONE', ( #662, #122687 ) ) ;
#121083=CARTESIAN_POINT ( 'NONE',  ( 5.649999999999934630, 2.500000000000000000, -1.818653347947325916 ) ) ;
#121084=CARTESIAN_POINT ( 'NONE',  ( -6.250000000000021316, 2.500000000000000000, -5.802370205355749988 ) ) ;
#121086=CIRCLE ( 'NONE', #93911, 0.06509327318403745899 ) ;
#121087=EDGE_LOOP ( 'NONE', ( #18125, #31495 ) ) ;
#121088=EDGE_LOOP ( 'NONE', ( #66178, #39232 ) ) ;
#121089=CARTESIAN_POINT ( 'NONE',  ( 14.59999999999989484, 2.500000000000000000, -0.6928203230275541413 ) ) ;
#121091=DIRECTION ( 'NONE',  ( -0.000000000000000000, -1.000000000000000000, -0.000000000000000000 ) ) ;
#121092=CARTESIAN_POINT ( 'NONE',  ( -5.400000000000019895, 12.50000000000000000, 3.702399969078682407 ) ) ;
#121093=DIRECTION ( 'NONE',  ( 0.000000000000000000, 0.000000000000000000, 1.000000000000000000 ) ) ;
#121094=EDGE_LOOP ( 'NONE', ( #71508, #44573, #114565, #5642 ) ) ;
#121095=DIRECTION ( 'NONE',  ( 0.000000000000000000, 0.000000000000000000, 1.000000000000000000 ) ) ;
#121096=CARTESIAN_POINT ( 'NONE',  ( -7.900000000000011013, 2.500000000000000000, 4.430127018922196847 ) ) ;
#121097=LINE ( 'NONE', #33385, #96690 ) ;
#121098=CARTESIAN_POINT ( 'NONE',  ( -12.89999999999999147, 12.50000000000000000, -4.330127018922198978 ) ) ;
#121099=DIRECTION ( 'NONE',  ( 0.000000000000000000, 0.000000000000000000, 1.000000000000000000 ) ) ;
#121100=AXIS2_PLACEMENT_3D ( 'NONE', #35504, #47901, #75402 ) ;
#121101=DIRECTION ( 'NONE',  ( 0.000000000000000000, 0.000000000000000000, 1.000000000000000000 ) ) ;
#121102=ORIENTED_EDGE ( 'NONE', *, *, #75888, .T. ) ;
#121103=EDGE_LOOP ( 'NONE', ( #51482, #71279, #127883, #3177 ) ) ;
#121104=CARTESIAN_POINT ( 'NONE',  ( -2.500000000000032419, 12.50000000000000000, -3.637306695894650055 ) ) ;
#121105=VERTEX_POINT ( 'NONE', #8901 ) ;
#121106=CARTESIAN_POINT ( 'NONE',  ( 9.799999999999918998, 2.500000000000000000, -0.2464101615137782308 ) ) ;
#121107=ORIENTED_EDGE ( 'NONE', *, *, #77988, .F. ) ;
#121108=ORIENTED_EDGE ( 'NONE', *, *, #54537, .F. ) ;
#121109=VERTEX_POINT ( 'NONE', #99889 ) ;
#121110=ADVANCED_FACE ( 'NONE', ( #8262 ), #44035, .T. ) ;
#121111=DIRECTION ( 'NONE',  ( -0.000000000000000000, 1.000000000000000000, -0.000000000000000000 ) ) ;
#121112=ADVANCED_FACE ( 'NONE', ( #89415 ), #86826, .T. ) ;
#121113=DIRECTION ( 'NONE',  ( 0.000000000000000000, 1.000000000000000000, 0.000000000000000000 ) ) ;
#121114=DIRECTION ( 'NONE',  ( 0.000000000000000000, -0.000000000000000000, 1.000000000000000000 ) ) ;
#121115=EDGE_CURVE ( 'NONE', #109940, #87133, #39843, .T. ) ;
#121116=CONICAL_SURFACE ( 'NONE', #106444, 0.1000000000000000472, 0.003490658503988666988 ) ;
#121117=CONICAL_SURFACE ( 'NONE', #66728, 0.09999999999999982514, 0.003490658503988666988 ) ;
#121118=CARTESIAN_POINT ( 'NONE',  ( 5.599999999999933031, 2.500000000000000000, 0.2464101615137735679 ) ) ;
#121119=DIRECTION ( 'NONE',  ( 0.000000000000000000, 1.000000000000000000, 0.000000000000000000 ) ) ;
#121120=CARTESIAN_POINT ( 'NONE',  ( 11.84999999999990372, 12.50000000000000000, 2.576566944158910744 ) ) ;
#121121=DIRECTION ( 'NONE',  ( 0.000000000000000000, 0.000000000000000000, -1.000000000000000000 ) ) ;
#121122=DIRECTION ( 'NONE',  ( 0.000000000000000000, 0.000000000000000000, 1.000000000000000000 ) ) ;
#121123=AXIS2_PLACEMENT_3D ( 'NONE', #5475, #36898, #97735 ) ;
#121124=EDGE_CURVE ( 'NONE', #14247, #78443, #10211, .T. ) ;
#121125=FACE_OUTER_BOUND ( 'NONE', #85831, .T. ) ;
#121126=EDGE_CURVE ( 'NONE', #74881, #66521, #125495, .T. ) ;
#121127=CIRCLE ( 'NONE', #8247, 9.000000000000001776 ) ;
#121128=ADVANCED_FACE ( 'NONE', ( #90041 ), #104569, .T. ) ;
#121129=ORIENTED_EDGE ( 'NONE', *, *, #93580, .F. ) ;
#121130=EDGE_CURVE ( 'NONE', #94015, #74258, #2159, .T. ) ;
#121131=DIRECTION ( 'NONE',  ( 0.000000000000000000, 0.000000000000000000, 1.000000000000000000 ) ) ;
#121132=ORIENTED_EDGE ( 'NONE', *, *, #73542, .F. ) ;
#121133=ORIENTED_EDGE ( 'NONE', *, *, #97026, .T. ) ;
#121134=CARTESIAN_POINT ( 'NONE',  ( 10.59999999999991260, 2.500000000000000000, -0.2464101615137783419 ) ) ;
#121135=CARTESIAN_POINT ( 'NONE',  ( -5.400000000000024336, 2.500000000000000000, -3.637306695894650055 ) ) ;
#121136=EDGE_CURVE ( 'NONE', #54303, #3400, #89978, .T. ) ;
#121137=DIRECTION ( 'NONE',  ( 0.000000000000000000, 0.000000000000000000, 1.000000000000000000 ) ) ;
#121138=CARTESIAN_POINT ( 'NONE',  ( -6.450000000000014388, 2.500000000000000000, 6.148780366869520897 ) ) ;
#121139=LINE ( 'NONE', #91681, #5117 ) ;
#121140=CARTESIAN_POINT ( 'NONE',  ( -7.950000000000009059, 12.50000000000000000, 6.430097255199259010 ) ) ;
#121141=CONICAL_SURFACE ( 'NONE', #68818, 0.1000000000000002554, 0.003490658503988666988 ) ;
#121142=ORIENTED_EDGE ( 'NONE', *, *, #75131, .T. ) ;
#121143=ORIENTED_EDGE ( 'NONE', *, *, #72304, .T. ) ;
#121144=VECTOR ( 'NONE', #71360, 1000.000000000000000 ) ;
#121145=AXIS2_PLACEMENT_3D ( 'NONE', #56104, #113100, #84930 ) ;
#121146=EDGE_LOOP ( 'NONE', ( #62538, #120772, #4976, #19896 ) ) ;
#121147=FACE_OUTER_BOUND ( 'NONE', #66885, .T. ) ;
#121148=VERTEX_POINT ( 'NONE', #103095 ) ;
#121149=EDGE_CURVE ( 'NONE', #108367, #28877, #33574, .T. ) ;
#121150=ORIENTED_EDGE ( 'NONE', *, *, #46756, .F. ) ;
#121151=DIRECTION ( 'NONE',  ( 0.000000000000000000, 0.000000000000000000, 1.000000000000000000 ) ) ;
#121152=VECTOR ( 'NONE', #36822, 1000.000000000000000 ) ;
#121153=FACE_OUTER_BOUND ( 'NONE', #54117, .T. ) ;
#121154=CIRCLE ( 'NONE', #18747, 0.1000000000000000056 ) ;
#121155=AXIS2_PLACEMENT_3D ( 'NONE', #105510, #51, #109364 ) ;
#121156=AXIS2_PLACEMENT_3D ( 'NONE', #76532, #116435, #106621 ) ;
#121157=CARTESIAN_POINT ( 'NONE',  ( -6.650000000000014566, 2.500000000000000000, 2.165063509461097713 ) ) ;
#121158=CARTESIAN_POINT ( 'NONE',  ( -9.400000000000007461, 2.500000000000000000, 0.3464101615137735735 ) ) ;
#121159=DIRECTION ( 'NONE',  ( 0.000000000000000000, 1.000000000000000000, 0.000000000000000000 ) ) ;
#121160=EDGE_LOOP ( 'NONE', ( #3884, #5172 ) ) ;
#121161=FACE_OUTER_BOUND ( 'NONE', #84354, .T. ) ;
#121162=DIRECTION ( 'NONE',  ( -0.000000000000000000, 1.000000000000000000, -0.000000000000000000 ) ) ;
#121163=FACE_OUTER_BOUND ( 'NONE', #6234, .T. ) ;
#121164=PLANE ( 'NONE',  #26346 ) ;
#121165=CIRCLE ( 'NONE', #37555, 0.06509327318403745899 ) ;
#121166=CARTESIAN_POINT ( 'NONE',  ( -9.999999999999969802, 2.500000000000000000, 0.09999999999999772959 ) ) ;
#121167=VERTEX_POINT ( 'NONE', #33095 ) ;
#121168=AXIS2_PLACEMENT_3D ( 'NONE', #88505, #117295, #67570 ) ;
#121169=EDGE_CURVE ( 'NONE', #89740, #92388, #54382, .T. ) ;
#121170=ORIENTED_EDGE ( 'NONE', *, *, #46806, .F. ) ;
#121171=ORIENTED_EDGE ( 'NONE', *, *, #22094, .F. ) ;
#121172=DIRECTION ( 'NONE',  ( 0.000000000000000000, 0.000000000000000000, 1.000000000000000000 ) ) ;
#121174=CIRCLE ( 'NONE', #119122, 0.06509327318403745899 ) ;
#121175=FACE_OUTER_BOUND ( 'NONE', #71410, .T. ) ;
#121176=CARTESIAN_POINT ( 'NONE',  ( 2.049999999999950084, 2.500000000000000000, -2.065063509461102065 ) ) ;
#121177=CIRCLE ( 'NONE', #60567, 0.09999999999999999167 ) ;
#121178=ORIENTED_EDGE ( 'NONE', *, *, #120757, .F. ) ;
#121179=DIRECTION ( 'NONE',  ( 0.000000000000000000, 0.000000000000000000, 1.000000000000000000 ) ) ;
#121180=CARTESIAN_POINT ( 'NONE',  ( -5.400000000000019895, 2.500000000000000000, 4.330127018922196314 ) ) ;
#121181=EDGE_CURVE ( 'NONE', #80836, #119345, #92633, .T. ) ;
#121182=DIRECTION ( 'NONE',  ( -4.274815082592931898E-19, -0.9999939076577903929, -0.003490651415223739937 ) ) ;
#121183=DIRECTION ( 'NONE',  ( -0.000000000000000000, -1.000000000000000000, -0.000000000000000000 ) ) ;
#121184=DIRECTION ( 'NONE',  ( 0.000000000000000000, 0.000000000000000000, 1.000000000000000000 ) ) ;
#121185=ORIENTED_EDGE ( 'NONE', *, *, #117516, .T. ) ;
#121186=ORIENTED_EDGE ( 'NONE', *, *, #125477, .F. ) ;
#121187=CARTESIAN_POINT ( 'NONE',  ( 26.75236858844773380, 2.962322775928817986, -2.722363799301888765 ) ) ;
#121188=LINE ( 'NONE', #128459, #51913 ) ;
#121189=DIRECTION ( 'NONE',  ( 0.000000000000000000, 0.000000000000000000, -1.000000000000000000 ) ) ;
#121190=DIRECTION ( 'NONE',  ( -0.000000000000000000, -1.000000000000000000, -0.000000000000000000 ) ) ;
#121191=VERTEX_POINT ( 'NONE', #61902 ) ;
#121192=VERTEX_POINT ( 'NONE', #22627 ) ;
#121193=FACE_OUTER_BOUND ( 'NONE', #43022, .T. ) ;
#121194=AXIS2_PLACEMENT_3D ( 'NONE', #121587, #50945, #21468 ) ;
#121195=CARTESIAN_POINT ( 'NONE',  ( 9.799999999999917222, 12.50000000000000000, 0.3464101615137735735 ) ) ;
#121196=DIRECTION ( 'NONE',  ( 0.000000000000000000, 1.000000000000000000, 0.000000000000000000 ) ) ;
#121197=DIRECTION ( 'NONE',  ( 0.000000000000000000, 1.000000000000000000, 0.000000000000000000 ) ) ;
#121198=VERTEX_POINT ( 'NONE', #11498 ) ;
#121199=DIRECTION ( 'NONE',  ( -4.274815082592931898E-19, -0.9999939076577903929, -0.003490651415223739937 ) ) ;
#121200=EDGE_CURVE ( 'NONE', #31897, #128741, #60669, .T. ) ;
#121201=CIRCLE ( 'NONE', #20863, 0.06509327318403745899 ) ;
#121202=CIRCLE ( 'NONE', #81509, 0.1000000000000000472 ) ;
#121203=LINE ( 'NONE', #71449, #97453 ) ;
#121204=ORIENTED_EDGE ( 'NONE', *, *, #90935, .F. ) ;
#121205=CARTESIAN_POINT ( 'NONE',  ( 15.19999999999989093, 12.50000000000000000, 0.2813168883297361700 ) ) ;
#121206=ORIENTED_EDGE ( 'NONE', *, *, #57557, .F. ) ;
#121207=CARTESIAN_POINT ( 'NONE',  ( -7.100000000000017408, 2.500000000000000000, -5.122947341949753763 ) ) ;
#121208=CONICAL_SURFACE ( 'NONE', #62742, 0.09999999999999982514, 0.003490658503988666988 ) ;
#121209=CIRCLE ( 'NONE', #110741, 0.1000000000000002554 ) ;
#121210=ORIENTED_EDGE ( 'NONE', *, *, #41468, .F. ) ;
#121211=ORIENTED_EDGE ( 'NONE', *, *, #81738, .F. ) ;
#121212=CARTESIAN_POINT ( 'NONE',  ( -9.350000000000008527, 2.500000000000000000, -6.941600689897073018 ) ) ;
#121213=CARTESIAN_POINT ( 'NONE',  ( 11.74779829714319135, 2.499999999999999556, -7.682567038344338073 ) ) ;
#121214=EDGE_CURVE ( 'NONE', #72985, #17629, #10822, .T. ) ;
#121215=ORIENTED_EDGE ( 'NONE', *, *, #59483, .T. ) ;
#121216=EDGE_CURVE ( 'NONE', #121192, #35232, #82172, .T. ) ;
#121217=ORIENTED_EDGE ( 'NONE', *, *, #16164, .T. ) ;
#121218=ADVANCED_FACE ( 'NONE', ( #91342 ), #71114, .T. ) ;
#121219=EDGE_CURVE ( 'NONE', #108239, #46118, #50780, .T. ) ;
#121220=FACE_OUTER_BOUND ( 'NONE', #105121, .T. ) ;
#121221=CARTESIAN_POINT ( 'NONE',  ( -10.60000000000000142, 12.50000000000000000, -0.3464101615137782364 ) ) ;
#121222=ORIENTED_EDGE ( 'NONE', *, *, #87530, .T. ) ;
#121225=EDGE_CURVE ( 'NONE', #65002, #99984, #62808, .T. ) ;
#121226=DIRECTION ( 'NONE',  ( 0.000000000000000000, 0.000000000000000000, -1.000000000000000000 ) ) ;
#121227=DIRECTION ( 'NONE',  ( 0.000000000000000000, 0.000000000000000000, -1.000000000000000000 ) ) ;
#121228=DIRECTION ( 'NONE',  ( 0.000000000000000000, 0.000000000000000000, 1.000000000000000000 ) ) ;
#121229=DIRECTION ( 'NONE',  ( 0.000000000000000000, -0.000000000000000000, 1.000000000000000000 ) ) ;
#121230=CARTESIAN_POINT ( 'NONE',  ( -12.94999999999999218, 2.500000000000000000, 2.165063509461101265 ) ) ;
#121231=ADVANCED_FACE ( 'NONE', ( #12763 ), #111635, .T. ) ;
#121232=EDGE_CURVE ( 'NONE', #54565, #9756, #100, .T. ) ;
#121233=VECTOR ( 'NONE', #110024, 1000.000000000000000 ) ;
#121234=EDGE_CURVE ( 'NONE', #60541, #20895, #122105, .T. ) ;
#121235=CIRCLE ( 'NONE', #25092, 0.09999999999999982514 ) ;
#121236=ORIENTED_EDGE ( 'NONE', *, *, #30447, .T. ) ;
#121237=EDGE_LOOP ( 'NONE', ( #54668, #125071, #122683, #117209 ) ) ;
#121238=DIRECTION ( 'NONE',  ( 0.000000000000000000, 1.000000000000000000, 0.000000000000000000 ) ) ;
#121239=ORIENTED_EDGE ( 'NONE', *, *, #8764, .T. ) ;
#121240=DIRECTION ( 'NONE',  ( -4.274815082592931898E-19, -0.9999939076577903929, -0.003490651415223739937 ) ) ;
#121241=DIRECTION ( 'NONE',  ( 0.000000000000000000, -0.000000000000000000, 1.000000000000000000 ) ) ;
#121242=DIRECTION ( 'NONE',  ( 0.000000000000000000, 1.000000000000000000, 0.000000000000000000 ) ) ;
#121243=ORIENTED_EDGE ( 'NONE', *, *, #17420, .F. ) ;
#121244=ORIENTED_EDGE ( 'NONE', *, *, #124648, .F. ) ;
#121246=FACE_BOUND ( 'NONE', #55573, .T. ) ;
#121247=EDGE_LOOP ( 'NONE', ( #53118, #108105, #70558, #117803 ) ) ;
#121248=ADVANCED_FACE ( 'NONE', ( #63172 ), #101817, .T. ) ;
#121249=DIRECTION ( 'NONE',  ( -0.000000000000000000, -1.000000000000000000, -0.000000000000000000 ) ) ;
#121250=DIRECTION ( 'NONE',  ( 0.000000000000000000, 1.000000000000000000, 0.000000000000000000 ) ) ;
#121251=VECTOR ( 'NONE', #115357, 1000.000000000000000 ) ;
#121252=CARTESIAN_POINT ( 'NONE',  ( 0.6499999999999561684, 12.50000000000000000, 1.753560074763284016 ) ) ;
#121253=CARTESIAN_POINT ( 'NONE',  ( 9.999999999999948486, 12.50000000000000000, 4.265033745738159077 ) ) ;
#121254=CARTESIAN_POINT ( 'NONE',  ( 3.349999999999941913, 12.50000000000000000, 5.737276932171707422 ) ) ;
#121255=DIRECTION ( 'NONE',  ( 0.000000000000000000, -0.000000000000000000, 1.000000000000000000 ) ) ;
#121256=FACE_OUTER_BOUND ( 'NONE', #124029, .T. ) ;
#121257=CARTESIAN_POINT ( 'NONE',  ( -1.250000000000001110, 2.500000000000000000, -6.595190528383302109 ) ) ;
#121258=FACE_OUTER_BOUND ( 'NONE', #47949, .T. ) ;
#121259=CARTESIAN_POINT ( 'NONE',  ( 4.999999999999935163, 2.500000000000000000, 3.737306695894644371 ) ) ;
#121260=AXIS2_PLACEMENT_3D ( 'NONE', #30614, #101914, #72459 ) ;
#121261=CARTESIAN_POINT ( 'NONE',  ( 10.19999999999991225, 2.500000000000000000, -4.676537180435978769 ) ) ;
#121262=AXIS2_PLACEMENT_3D ( 'NONE', #25702, #57760, #125828 ) ;
#121263=ORIENTED_EDGE ( 'NONE', *, *, #3955, .F. ) ;
#121264=EDGE_LOOP ( 'NONE', ( #123502, #112744, #75210, #61951 ) ) ;
#121265=ORIENTED_EDGE ( 'NONE', *, *, #60418, .T. ) ;
#121266=ORIENTED_EDGE ( 'NONE', *, *, #18339, .T. ) ;
#121267=DIRECTION ( 'NONE',  ( 0.000000000000000000, 0.000000000000000000, -1.000000000000000000 ) ) ;
#121268=CARTESIAN_POINT ( 'NONE',  ( 8.549999999999922551, 12.50000000000000000, 2.446380397790835826 ) ) ;
#121269=ORIENTED_EDGE ( 'NONE', *, *, #78188, .T. ) ;
#121270=ORIENTED_EDGE ( 'NONE', *, *, #84749, .F. ) ;
#121271=EDGE_LOOP ( 'NONE', ( #84807, #120112 ) ) ;
#121274=CARTESIAN_POINT ( 'NONE',  ( 2.299999999999949640, 2.500000000000000000, -4.676537180435977881 ) ) ;
#121275=CARTESIAN_POINT ( 'NONE',  ( -1.450000000000036371, 12.50000000000000000, 6.841600689897072485 ) ) ;
#121276=DIRECTION ( 'NONE',  ( 0.000000000000000000, -0.000000000000000000, 1.000000000000000000 ) ) ;
#121277=DIRECTION ( 'NONE',  ( 0.000000000000000000, 0.000000000000000000, -1.000000000000000000 ) ) ;
#121278=CIRCLE ( 'NONE', #6319, 0.1000000000000002554 ) ;
#121279=CARTESIAN_POINT ( 'NONE',  ( 8.349999999999923261, 12.50000000000000000, -6.430097255199264339 ) ) ;
#121280=DIRECTION ( 'NONE',  ( -0.000000000000000000, 1.000000000000000000, -0.000000000000000000 ) ) ;
#121281=VERTEX_POINT ( 'NONE', #93925 ) ;
#121282=CARTESIAN_POINT ( 'NONE',  ( 3.149999999999946176, 2.500000000000000000, -6.841600689897077814 ) ) ;
#121283=ORIENTED_EDGE ( 'NONE', *, *, #127164, .F. ) ;
#121284=EDGE_CURVE ( 'NONE', #72341, #86064, #37679, .T. ) ;
#121285=ORIENTED_EDGE ( 'NONE', *, *, #45549, .T. ) ;
#121286=ORIENTED_EDGE ( 'NONE', *, *, #42776, .T. ) ;
#121287=EDGE_CURVE ( 'NONE', #83886, #89736, #87827, .T. ) ;
#121288=DIRECTION ( 'NONE',  ( 0.000000000000000000, 0.000000000000000000, 1.000000000000000000 ) ) ;
#121291=ORIENTED_EDGE ( 'NONE', *, *, #52438, .T. ) ;
#121292=ORIENTED_EDGE ( 'NONE', *, *, #67109, .F. ) ;
#121294=EDGE_CURVE ( 'NONE', #95328, #97364, #36310, .T. ) ;
#121295=FACE_OUTER_BOUND ( 'NONE', #87082, .T. ) ;
#121296=FACE_OUTER_BOUND ( 'NONE', #53861, .T. ) ;
#121297=DIRECTION ( 'NONE',  ( 0.000000000000000000, 1.000000000000000000, 0.000000000000000000 ) ) ;
#121298=CIRCLE ( 'NONE', #25143, 0.06509327318403745899 ) ;
#121299=DIRECTION ( 'NONE',  ( -0.000000000000000000, 1.000000000000000000, -0.000000000000000000 ) ) ;
#121300=AXIS2_PLACEMENT_3D ( 'NONE', #16773, #5034, #105177 ) ;
#121302=VERTEX_POINT ( 'NONE', #113562 ) ;
#121303=DIRECTION ( 'NONE',  ( 0.000000000000000000, 1.000000000000000000, 0.000000000000000000 ) ) ;
#121304=AXIS2_PLACEMENT_3D ( 'NONE', #32345, #50665, #9457 ) ;
#121305=VECTOR ( 'NONE', #79528, 1000.000000000000000 ) ;
#121306=ORIENTED_EDGE ( 'NONE', *, *, #60052, .F. ) ;
#121307=CARTESIAN_POINT ( 'NONE',  ( 6.249999999999965361, 2.500000000000000000, 2.165063509461097713 ) ) ;
#121308=ORIENTED_EDGE ( 'NONE', *, *, #29001, .T. ) ;
#121309=DIRECTION ( 'NONE',  ( 0.000000000000000000, 0.000000000000000000, 1.000000000000000000 ) ) ;
#121310=EDGE_LOOP ( 'NONE', ( #57510, #32407 ) ) ;
#121311=DIRECTION ( 'NONE',  ( -0.000000000000000000, -1.000000000000000000, -0.000000000000000000 ) ) ;
#121312=DIRECTION ( 'NONE',  ( 0.000000000000000000, 0.000000000000000000, 1.000000000000000000 ) ) ;
#121313=ORIENTED_EDGE ( 'NONE', *, *, #102573, .F. ) ;
#121314=ORIENTED_EDGE ( 'NONE', *, *, #47287, .T. ) ;
#121316=DIRECTION ( 'NONE',  ( -0.000000000000000000, -1.000000000000000000, -0.000000000000000000 ) ) ;
#121318=DIRECTION ( 'NONE',  ( 0.000000000000000000, 0.000000000000000000, 1.000000000000000000 ) ) ;
#121319=DIRECTION ( 'NONE',  ( 0.000000000000000000, 0.000000000000000000, -1.000000000000000000 ) ) ;
#121320=ORIENTED_EDGE ( 'NONE', *, *, #43037, .F. ) ;
#121321=LINE ( 'NONE', #905, #23652 ) ;
#121322=ORIENTED_EDGE ( 'NONE', *, *, #100279, .T. ) ;
#121323=DIRECTION ( 'NONE',  ( -0.000000000000000000, -1.000000000000000000, -0.000000000000000000 ) ) ;
#121324=AXIS2_PLACEMENT_3D ( 'NONE', #3283, #83146, #33406 ) ;
#121325=DIRECTION ( 'NONE',  ( -4.274815082592931898E-19, -0.9999939076577903929, -0.003490651415223739937 ) ) ;
#121326=VECTOR ( 'NONE', #62064, 1000.000000000000000 ) ;
#121327=EDGE_CURVE ( 'NONE', #58914, #8254, #24538, .T. ) ;
#121328=CARTESIAN_POINT ( 'NONE',  ( 11.44999999999990514, 2.500000000000000000, 2.511473670974873507 ) ) ;
#121329=DIRECTION ( 'NONE',  ( 0.000000000000000000, 1.000000000000000000, 0.000000000000000000 ) ) ;
#121330=DIRECTION ( 'NONE',  ( 0.000000000000000000, 0.000000000000000000, 1.000000000000000000 ) ) ;
#121331=EDGE_CURVE ( 'NONE', #49253, #37140, #102593, .T. ) ;
#121332=DIRECTION ( 'NONE',  ( 0.000000000000000000, 0.000000000000000000, 1.000000000000000000 ) ) ;
#121333=CARTESIAN_POINT ( 'NONE',  ( 10.39999999999991154, 2.500000000000000000, 3.637306695894644726 ) ) ;
#121334=ORIENTED_EDGE ( 'NONE', *, *, #109256, .T. ) ;
#121335=VECTOR ( 'NONE', #73690, 1000.000000000000000 ) ;
#121336=CARTESIAN_POINT ( 'NONE',  ( -12.69999999999999041, 12.50000000000000000, 3.983716857408420964 ) ) ;
#121337=DIRECTION ( 'NONE',  ( 0.000000000000000000, 1.000000000000000000, 0.000000000000000000 ) ) ;
#121338=FACE_OUTER_BOUND ( 'NONE', #110915, .T. ) ;
#121339=EDGE_CURVE ( 'NONE', #29412, #115297, #43552, .T. ) ;
#121340=ORIENTED_EDGE ( 'NONE', *, *, #66828, .T. ) ;
#121341=DIRECTION ( 'NONE',  ( 0.000000000000000000, -0.9999939076577903929, 0.003490651415223739937 ) ) ;
#121342=AXIS2_PLACEMENT_3D ( 'NONE', #9934, #11212, #88482 ) ;
#121343=CIRCLE ( 'NONE', #123400, 0.09999999999999982514 ) ;
#121344=EDGE_LOOP ( 'NONE', ( #26464, #89232, #56227, #42009 ) ) ;
#121345=ORIENTED_EDGE ( 'NONE', *, *, #81076, .F. ) ;
#121346=DIRECTION ( 'NONE',  ( -0.000000000000000000, -1.000000000000000000, -0.000000000000000000 ) ) ;
#121347=ORIENTED_EDGE ( 'NONE', *, *, #82711, .F. ) ;
#121348=CARTESIAN_POINT ( 'NONE',  ( 16.86689433361074819, -2.548103353434854057, -5.776876940651522574 ) ) ;
#121349=DIRECTION ( 'NONE',  ( -0.000000000000000000, 1.000000000000000000, -0.000000000000000000 ) ) ;
#121350=AXIS2_PLACEMENT_3D ( 'NONE', #15734, #5903, #45863 ) ;
#121351=ORIENTED_EDGE ( 'NONE', *, *, #124185, .T. ) ;
#121352=DIRECTION ( 'NONE',  ( -0.000000000000000000, -1.000000000000000000, -0.000000000000000000 ) ) ;
#121354=CARTESIAN_POINT ( 'NONE',  ( 4.199999999999941558, 12.50000000000000000, -4.330127018922201643 ) ) ;
#121355=AXIS2_PLACEMENT_3D ( 'NONE', #29789, #18675, #28506 ) ;
#121357=EDGE_CURVE ( 'NONE', #66637, #69877, #23172, .T. ) ;
#121358=ORIENTED_EDGE ( 'NONE', *, *, #59790, .T. ) ;
#121359=VERTEX_POINT ( 'NONE', #55925 ) ;
#121360=CARTESIAN_POINT ( 'NONE',  ( -1.050000000000037792, 12.50000000000000000, 6.083687093685482772 ) ) ;
#121361=CARTESIAN_POINT ( 'NONE',  ( -2.499999999999996447, 2.500000000000000000, 4.230127018922196669 ) ) ;
#121362=DIRECTION ( 'NONE',  ( 0.000000000000000000, 0.000000000000000000, -1.000000000000000000 ) ) ;
#121363=ADVANCED_FACE ( 'NONE', ( #84748 ), #94556, .T. ) ;
#121364=ADVANCED_FACE ( 'NONE', ( #95860 ), #37765, .T. ) ;
#121365=FACE_BOUND ( 'NONE', #9994, .T. ) ;
#121366=ORIENTED_EDGE ( 'NONE', *, *, #54007, .T. ) ;
#121367=EDGE_CURVE ( 'NONE', #113231, #118968, #14050, .T. ) ;
#121368=EDGE_CURVE ( 'NONE', #128991, #38337, #45485, .T. ) ;
#121369=CARTESIAN_POINT ( 'NONE',  ( -0.4000000000000401013, 2.500000000000000000, -3.737306695894649700 ) ) ;
#121370=DIRECTION ( 'NONE',  ( 0.000000000000000000, -0.9999939076577903929, 0.003490651415223739937 ) ) ;
#121371=ORIENTED_EDGE ( 'NONE', *, *, #51526, .F. ) ;
#121372=DIRECTION ( 'NONE',  ( -0.000000000000000000, 1.000000000000000000, -0.000000000000000000 ) ) ;
#121373=DIRECTION ( 'NONE',  ( 0.000000000000000000, 0.000000000000000000, 1.000000000000000000 ) ) ;
#121374=EDGE_CURVE ( 'NONE', #65870, #10740, #183, .T. ) ;
#121375=AXIS2_PLACEMENT_3D ( 'NONE', #73624, #64454, #103748 ) ;
#121376=CARTESIAN_POINT ( 'NONE',  ( -12.69999999999999218, 12.50000000000000000, -0.3464101615137741286 ) ) ;
#121377=CARTESIAN_POINT ( 'NONE',  ( -9.200000000000006395, 12.50000000000000000, 0.06509327318403504425 ) ) ;
#121378=CARTESIAN_POINT ( 'NONE',  ( -9.150000000000009237, 2.500000000000000000, 2.065063509461097624 ) ) ;
#121379=AXIS2_PLACEMENT_3D ( 'NONE', #1522, #40838, #111479 ) ;
#121380=EDGE_CURVE ( 'NONE', #91731, #118811, #67063, .T. ) ;
#121381=DIRECTION ( 'NONE',  ( 0.000000000000000000, 1.000000000000000000, 0.000000000000000000 ) ) ;
#121382=DIRECTION ( 'NONE',  ( -0.000000000000000000, 1.000000000000000000, -0.000000000000000000 ) ) ;
#121383=EDGE_CURVE ( 'NONE', #127901, #91908, #39923, .T. ) ;
#121384=CIRCLE ( 'NONE', #8502, 0.06509327318403745899 ) ;
#121385=EDGE_CURVE ( 'NONE', #59408, #125792, #106795, .T. ) ;
#121386=EDGE_LOOP ( 'NONE', ( #19212, #32568 ) ) ;
#121387=ORIENTED_EDGE ( 'NONE', *, *, #80130, .F. ) ;
#121388=ORIENTED_EDGE ( 'NONE', *, *, #45686, .T. ) ;
#121389=ORIENTED_EDGE ( 'NONE', *, *, #105596, .F. ) ;
#121390=CARTESIAN_POINT ( 'NONE',  ( -0.6500000000000398792, 12.50000000000000000, -2.576566944158915184 ) ) ;
#121391=AXIS2_PLACEMENT_3D ( 'NONE', #20671, #60608, #21972 ) ;
#121392=CARTESIAN_POINT ( 'NONE',  ( -1.900000000000034994, 12.50000000000000000, -4.611443907251940644 ) ) ;
#121393=VERTEX_POINT ( 'NONE', #25828 ) ;
#121394=ADVANCED_FACE ( 'NONE', ( #6167 ), #15338, .T. ) ;
#121395=FACE_BOUND ( 'NONE', #114015, .T. ) ;
#121396=ADVANCED_FACE ( 'NONE', ( #35651 ), #75558, .T. ) ;
#121397=CARTESIAN_POINT ( 'NONE',  ( 13.74999999999993072, 2.500000000000000000, -2.065063509461102065 ) ) ;
#121398=DIRECTION ( 'NONE',  ( 0.000000000000000000, 0.000000000000000000, 1.000000000000000000 ) ) ;
#121399=CARTESIAN_POINT ( 'NONE',  ( 4.999999999999935163, 12.50000000000000000, 3.637306695894644726 ) ) ;
#121400=LINE ( 'NONE', #42212, #113959 ) ;
#121401=DIRECTION ( 'NONE',  ( 0.000000000000000000, 1.000000000000000000, 0.000000000000000000 ) ) ;
#121402=DIRECTION ( 'NONE',  ( 0.000000000000000000, 0.000000000000000000, 1.000000000000000000 ) ) ;
#121403=DIRECTION ( 'NONE',  ( 0.000000000000000000, 0.000000000000000000, -1.000000000000000000 ) ) ;
#121404=DIRECTION ( 'NONE',  ( -4.274815082592931898E-19, -0.9999939076577903929, -0.003490651415223739937 ) ) ;
#121405=CARTESIAN_POINT ( 'NONE',  ( -5.000000000000026645, 12.50000000000000000, -3.637306695894650055 ) ) ;
#121406=ORIENTED_EDGE ( 'NONE', *, *, #76448, .T. ) ;
#121407=ORIENTED_EDGE ( 'NONE', *, *, #90834, .T. ) ;
#121408=VERTEX_POINT ( 'NONE', #80577 ) ;
#121409=ORIENTED_EDGE ( 'NONE', *, *, #39213, .F. ) ;
#121410=ORIENTED_EDGE ( 'NONE', *, *, #24004, .F. ) ;
#121411=EDGE_LOOP ( 'NONE', ( #123722, #104802, #99937, #88787 ) ) ;
#121412=DIRECTION ( 'NONE',  ( -0.000000000000000000, -1.000000000000000000, -0.000000000000000000 ) ) ;
#121414=CONICAL_SURFACE ( 'NONE', #48259, 0.1000000000000002554, 0.003490658503988666988 ) ;
#121415=AXIS2_PLACEMENT_3D ( 'NONE', #36477, #107769, #85549 ) ;
#121416=LINE ( 'NONE', #10792, #72859 ) ;
#121417=CARTESIAN_POINT ( 'NONE',  ( 15.50668944026786278, -2.500000000000065281, 6.997696164093700766 ) ) ;
#121418=CARTESIAN_POINT ( 'NONE',  ( -7.500000000000001776, 2.500000000000000000, 1.734723475976807094E-15 ) ) ;
#121419=DIRECTION ( 'NONE',  ( -0.000000000000000000, 1.000000000000000000, -0.000000000000000000 ) ) ;
#121420=ORIENTED_EDGE ( 'NONE', *, *, #56452, .F. ) ;
#121421=DIRECTION ( 'NONE',  ( 0.000000000000000000, 1.000000000000000000, 0.000000000000000000 ) ) ;
#121422=VECTOR ( 'NONE', #24917, 1000.000000000000000 ) ;
#121423=ORIENTED_EDGE ( 'NONE', *, *, #17549, .T. ) ;
#121424=EDGE_CURVE ( 'NONE', #15508, #23590, #4371, .T. ) ;
#121425=EDGE_LOOP ( 'NONE', ( #52923, #86577 ) ) ;
#121426=FACE_OUTER_BOUND ( 'NONE', #48078, .T. ) ;
#121427=EDGE_CURVE ( 'NONE', #125357, #23344, #38740, .T. ) ;
#121428=LINE ( 'NONE', #1018, #40646 ) ;
#121429=DIRECTION ( 'NONE',  ( 0.000000000000000000, 1.000000000000000000, 0.000000000000000000 ) ) ;
#121430=EDGE_LOOP ( 'NONE', ( #126290, #47206, #52682, #107585 ) ) ;
#121431=ORIENTED_EDGE ( 'NONE', *, *, #10919, .T. ) ;
#121432=CIRCLE ( 'NONE', #81721, 0.06509327318403745899 ) ;
#121433=DIRECTION ( 'NONE',  ( 0.000000000000000000, 0.000000000000000000, -1.000000000000000000 ) ) ;
#121434=CONICAL_SURFACE ( 'NONE', #8552, 0.1000000000000002554, 0.003490658503988666988 ) ;
#121435=DIRECTION ( 'NONE',  ( 0.000000000000000000, 0.000000000000000000, -1.000000000000000000 ) ) ;
#121436=CARTESIAN_POINT ( 'NONE',  ( 10.39999999999991154, 2.500000000000000000, -3.637306695894650055 ) ) ;
#121437=CARTESIAN_POINT ( 'NONE',  ( -9.999999999999969802, 2.500000000000000000, -2.276824562219559311E-15 ) ) ;
#121438=VERTEX_POINT ( 'NONE', #40011 ) ;
#121439=CARTESIAN_POINT ( 'NONE',  ( -10.45000000000000107, 12.50000000000000000, 2.165063509461097713 ) ) ;
#121440=AXIS2_PLACEMENT_3D ( 'NONE', #19457, #30593, #78404 ) ;
#121441=ORIENTED_EDGE ( 'NONE', *, *, #101552, .F. ) ;
#121442=CARTESIAN_POINT ( 'NONE',  ( 13.39053294304968134, -2.500000000000001332, 7.037281287790809081 ) ) ;
#121443=EDGE_LOOP ( 'NONE', ( #89081, #108368, #96998, #8223 ) ) ;
#121444=CARTESIAN_POINT ( 'NONE',  ( 17.50000000000000000, 2.499999999999999556, 2.333333333333335702 ) ) ;
#121445=CARTESIAN_POINT ( 'NONE',  ( 26.74601956401501468, -2.978655701349517848, 2.722801865438416069 ) ) ;
#121446=CONICAL_SURFACE ( 'NONE', #119385, 0.1000000000000000472, 0.003490658503988666988 ) ;
#121447=LINE ( 'NONE', #52085, #107536 ) ;
#121448=CARTESIAN_POINT ( 'NONE',  ( 0.5999999999999551248, 2.500000000000000000, -4.676537180435978769 ) ) ;
#121449=CARTESIAN_POINT ( 'NONE',  ( -13.34999999999999076, 12.50000000000000000, -2.165063509461099489 ) ) ;
#121450=EDGE_LOOP ( 'NONE', ( #53571, #2792 ) ) ;
#121451=LINE ( 'NONE', #11510, #30058 ) ;
#121452=DIRECTION ( 'NONE',  ( 0.000000000000000000, 1.000000000000000000, 0.000000000000000000 ) ) ;
#121453=VERTEX_POINT ( 'NONE', #79921 ) ;
#121454=ORIENTED_EDGE ( 'NONE', *, *, #115411, .T. ) ;
#121455=EDGE_LOOP ( 'NONE', ( #39024, #32887 ) ) ;
#121456=CARTESIAN_POINT ( 'NONE',  ( 2.500000000000002220, 2.750000000000000000, 10.00000000000000178 ) ) ;
#121457=FACE_OUTER_BOUND ( 'NONE', #74745, .T. ) ;
#121459=DIRECTION ( 'NONE',  ( 0.000000000000000000, 0.000000000000000000, 1.000000000000000000 ) ) ;
#121460=DIRECTION ( 'NONE',  ( 0.000000000000000000, 1.000000000000000000, 0.000000000000000000 ) ) ;
#121461=ADVANCED_FACE ( 'NONE', ( #9252 ), #21034, .T. ) ;
#121462=DIRECTION ( 'NONE',  ( 0.000000000000000000, 0.000000000000000000, 1.000000000000000000 ) ) ;
#121463=CARTESIAN_POINT ( 'NONE',  ( 11.64999999999990266, 12.50000000000000000, -6.495190528383302464 ) ) ;
#121465=CIRCLE ( 'NONE', #12792, 0.1000000000000000472 ) ;
#121466=AXIS2_PLACEMENT_3D ( 'NONE', #6025, #45981, #106185 ) ;
#121467=AXIS2_PLACEMENT_3D ( 'NONE', #84744, #105012, #124679 ) ;
#121469=EDGE_LOOP ( 'NONE', ( #53312, #48464 ) ) ;
#121470=DIRECTION ( 'NONE',  ( -0.000000000000000000, -1.000000000000000000, -0.000000000000000000 ) ) ;
#121471=AXIS2_PLACEMENT_3D ( 'NONE', #127882, #78153, #48686 ) ;
#121472=EDGE_CURVE ( 'NONE', #103811, #124333, #4278, .T. ) ;
#121473=DIRECTION ( 'NONE',  ( -0.000000000000000000, 1.000000000000000000, -0.000000000000000000 ) ) ;
#121474=EDGE_CURVE ( 'NONE', #81857, #124173, #59000, .T. ) ;
#121475=DIRECTION ( 'NONE',  ( -0.000000000000000000, -1.000000000000000000, -0.000000000000000000 ) ) ;
#121476=CARTESIAN_POINT ( 'NONE',  ( 17.50000000000000000, -2.500000000000000000, 0.000000000000000000 ) ) ;
#121477=VERTEX_POINT ( 'NONE', #60307 ) ;
#121478=DIRECTION ( 'NONE',  ( -0.000000000000000000, 1.000000000000000000, -0.000000000000000000 ) ) ;
#121479=DIRECTION ( 'NONE',  ( 0.000000000000000000, 1.000000000000000000, 0.000000000000000000 ) ) ;
#121480=CARTESIAN_POINT ( 'NONE',  ( 6.899999999999928413, 2.500000000000000000, 4.576537180435972019 ) ) ;
#121481=VERTEX_POINT ( 'NONE', #28900 ) ;
#121482=EDGE_CURVE ( 'NONE', #64399, #33567, #100831, .T. ) ;
#121483=ORIENTED_EDGE ( 'NONE', *, *, #816, .T. ) ;
#121484=DIRECTION ( 'NONE',  ( 0.000000000000000000, -0.9999939076577903929, 0.003490651415223739937 ) ) ;
#121485=ORIENTED_EDGE ( 'NONE', *, *, #104526, .F. ) ;
#121486=VERTEX_POINT ( 'NONE', #18423 ) ;
#121487=DIRECTION ( 'NONE',  ( 0.000000000000000000, 0.000000000000000000, 1.000000000000000000 ) ) ;
#121488=DIRECTION ( 'NONE',  ( -0.000000000000000000, 1.000000000000000000, -0.000000000000000000 ) ) ;
#121489=LINE ( 'NONE', #22684, #69384 ) ;
#121490=CARTESIAN_POINT ( 'NONE',  ( -7.900000000000014566, 2.500000000000000000, -0.5928203230275541635 ) ) ;
#121491=CIRCLE ( 'NONE', #113101, 0.06509327318403745899 ) ;
#121492=EDGE_LOOP ( 'NONE', ( #24993, #28667 ) ) ;
#121493=AXIS2_PLACEMENT_3D ( 'NONE', #50009, #109556, #108886 ) ;
#121494=DIRECTION ( 'NONE',  ( 0.000000000000000000, 0.000000000000000000, -1.000000000000000000 ) ) ;
#121495=ORIENTED_EDGE ( 'NONE', *, *, #49351, .T. ) ;
#121496=DIRECTION ( 'NONE',  ( -4.274815082592931898E-19, -0.9999939076577903929, -0.003490651415223739937 ) ) ;
#121497=CARTESIAN_POINT ( 'NONE',  ( 2.499999999999947153, 2.500000000000000000, -3.637306695894650055 ) ) ;
#121498=AXIS2_PLACEMENT_3D ( 'NONE', #32307, #1513, #72213 ) ;
#121499=VERTEX_POINT ( 'NONE', #89103 ) ;
#121500=VECTOR ( 'NONE', #39871, 1000.000000000000000 ) ;
#121501=EDGE_CURVE ( 'NONE', #6155, #127958, #71205, .T. ) ;
#121502=VERTEX_POINT ( 'NONE', #120495 ) ;
#121503=ORIENTED_EDGE ( 'NONE', *, *, #126123, .F. ) ;
#121504=ORIENTED_EDGE ( 'NONE', *, *, #116498, .F. ) ;
#121506=CARTESIAN_POINT ( 'NONE',  ( -8.750000000000010658, 2.500000000000000000, -7.288010851410849256 ) ) ;
#121507=CARTESIAN_POINT ( 'NONE',  ( -6.900000000000015454, 2.500000000000000000, 3.883716857408420431 ) ) ;
#121508=EDGE_CURVE ( 'NONE', #115621, #20962, #50454, .T. ) ;
#121509=FACE_BOUND ( 'NONE', #89174, .T. ) ;
#121510=EDGE_LOOP ( 'NONE', ( #97495, #126048, #971, #86924 ) ) ;
#121511=CARTESIAN_POINT ( 'NONE',  ( -0.6000000000000383915, 2.500000000000000000, -3.983716857408426293 ) ) ;
#121513=EDGE_CURVE ( 'NONE', #49354, #102850, #64936, .T. ) ;
#121514=DIRECTION ( 'NONE',  ( 0.000000000000000000, -0.000000000000000000, 1.000000000000000000 ) ) ;
#121515=DIRECTION ( 'NONE',  ( 0.000000000000000000, -0.000000000000000000, 1.000000000000000000 ) ) ;
#121516=AXIS2_PLACEMENT_3D ( 'NONE', #4433, #105892, #74500 ) ;
#121517=AXIS2_PLACEMENT_3D ( 'NONE', #77565, #26552, #58596 ) ;
#121518=CIRCLE ( 'NONE', #83965, 0.1000000000000002554 ) ;
#121519=ADVANCED_FACE ( 'NONE', ( #90368 ), #14741, .T. ) ;
#121520=FACE_OUTER_BOUND ( 'NONE', #22902, .T. ) ;
#121521=EDGE_CURVE ( 'NONE', #90643, #34472, #40669, .T. ) ;
#121522=DIRECTION ( 'NONE',  ( -0.000000000000000000, -1.000000000000000000, -0.000000000000000000 ) ) ;
#121524=EDGE_CURVE ( 'NONE', #56692, #49433, #77470, .T. ) ;
#121525=DIRECTION ( 'NONE',  ( 0.000000000000000000, 1.000000000000000000, 0.000000000000000000 ) ) ;
#121526=CIRCLE ( 'NONE', #69204, 0.1000000000000000472 ) ;
#121527=EDGE_CURVE ( 'NONE', #120101, #40494, #20995, .T. ) ;
#121528=LINE ( 'NONE', #111051, #78687 ) ;
#121529=EDGE_CURVE ( 'NONE', #69367, #4802, #123519, .T. ) ;
#121530=ORIENTED_EDGE ( 'NONE', *, *, #125665, .T. ) ;
#121531=CIRCLE ( 'NONE', #92295, 0.06509327318403745899 ) ;
#121532=CIRCLE ( 'NONE', #67137, 0.06509327318403745899 ) ;
#121533=VERTEX_POINT ( 'NONE', #99579 ) ;
#121534=ORIENTED_EDGE ( 'NONE', *, *, #3192, .T. ) ;
#121535=VERTEX_POINT ( 'NONE', #8579 ) ;
#121537=CARTESIAN_POINT ( 'NONE',  ( -2.500000000000032419, 12.50000000000000000, 0.7579135962115869374 ) ) ;
#121538=DIRECTION ( 'NONE',  ( 0.000000000000000000, 0.000000000000000000, 1.000000000000000000 ) ) ;
#121540=FACE_BOUND ( 'NONE', #59162, .T. ) ;
#121543=VERTEX_POINT ( 'NONE', #106320 ) ;
#121544=CARTESIAN_POINT ( 'NONE',  ( 4.599999999999938360, 2.500000000000000000, -2.276824562219559311E-15 ) ) ;
#121545=DIRECTION ( 'NONE',  ( -0.000000000000000000, 1.000000000000000000, -0.000000000000000000 ) ) ;
#121546=CARTESIAN_POINT ( 'NONE',  ( -8.100000000000010303, 12.50000000000000000, 4.676537180435972552 ) ) ;
#121548=ORIENTED_EDGE ( 'NONE', *, *, #55463, .T. ) ;
#121549=DIRECTION ( 'NONE',  ( 0.000000000000000000, -0.000000000000000000, 1.000000000000000000 ) ) ;
#121550=ORIENTED_EDGE ( 'NONE', *, *, #4064, .T. ) ;
#121552=CIRCLE ( 'NONE', #111074, 0.1000000000000000472 ) ;
#121553=ORIENTED_EDGE ( 'NONE', *, *, #119189, .T. ) ;
#121554=AXIS2_PLACEMENT_3D ( 'NONE', #129399, #40363, #128086 ) ;
#121555=CARTESIAN_POINT ( 'NONE',  ( 8.749999999999921840, 2.500000000000000000, -5.802370205355749988 ) ) ;
#121556=AXIS2_PLACEMENT_3D ( 'NONE', #114685, #45972, #14545 ) ;
#121557=CARTESIAN_POINT ( 'NONE',  ( 5.649999999999934630, 12.50000000000000000, -1.818653347947325916 ) ) ;
#121558=EDGE_LOOP ( 'NONE', ( #105762, #34136, #25696, #87168 ) ) ;
#121559=CARTESIAN_POINT ( 'NONE',  ( 9.799999999999913669, 2.500000000000000000, -3.983716857408426293 ) ) ;
#121560=CARTESIAN_POINT ( 'NONE',  ( 15.83209681635555022, 1.499999999999999556, -5.404881881984138658 ) ) ;
#121562=CARTESIAN_POINT ( 'NONE',  ( -13.14999999999999147, 2.500000000000000000, 1.818653347947325472 ) ) ;
#121563=CONICAL_SURFACE ( 'NONE', #16976, 0.1000000000000002554, 0.003490658503988666988 ) ;
#121564=DIRECTION ( 'NONE',  ( 0.000000000000000000, 0.000000000000000000, -1.000000000000000000 ) ) ;
#121566=VERTEX_POINT ( 'NONE', #48534 ) ;
#121567=AXIS2_PLACEMENT_3D ( 'NONE', #116251, #26597, #124144 ) ;
#121568=CARTESIAN_POINT ( 'NONE',  ( -12.49999999999995914, 2.500000000000000000, -4.430127018922199511 ) ) ;
#121569=ORIENTED_EDGE ( 'NONE', *, *, #45020, .T. ) ;
#121570=CARTESIAN_POINT ( 'NONE',  ( 3.749999999999975131, 12.50000000000000000, 6.430097255199259010 ) ) ;
#121571=CIRCLE ( 'NONE', #109042, 0.1000000000000000472 ) ;
#121572=EDGE_LOOP ( 'NONE', ( #63230, #25821 ) ) ;
#121573=EDGE_CURVE ( 'NONE', #129420, #65503, #18961, .T. ) ;
#121574=DIRECTION ( 'NONE',  ( 0.000000000000000000, -0.000000000000000000, 1.000000000000000000 ) ) ;
#121575=VERTEX_POINT ( 'NONE', #4543 ) ;
#121576=FACE_OUTER_BOUND ( 'NONE', #38804, .T. ) ;
#121577=CARTESIAN_POINT ( 'NONE',  ( 13.34999999999990017, 12.50000000000000000, 2.857883832488649301 ) ) ;
#121578=CARTESIAN_POINT ( 'NONE',  ( -5.600000000000020073, 2.500000000000000000, 0.4464101615137736623 ) ) ;
#121579=CARTESIAN_POINT ( 'NONE',  ( 6.899999999999928413, 12.50000000000000000, 4.676537180435972552 ) ) ;
#121580=CARTESIAN_POINT ( 'NONE',  ( -7.900000000000011013, 12.50000000000000000, 3.702399969078682407 ) ) ;
#121581=ORIENTED_EDGE ( 'NONE', *, *, #53385, .T. ) ;
#121582=ORIENTED_EDGE ( 'NONE', *, *, #109636, .T. ) ;
#121583=EDGE_CURVE ( 'NONE', #68393, #45961, #13091, .T. ) ;
#121584=ORIENTED_EDGE ( 'NONE', *, *, #25165, .F. ) ;
#121585=CARTESIAN_POINT ( 'NONE',  ( -3.150000000000030109, 2.500000000000000000, 1.818653347947321475 ) ) ;
#121586=DIRECTION ( 'NONE',  ( 0.000000000000000000, 1.000000000000000000, 0.000000000000000000 ) ) ;
#121587=CARTESIAN_POINT ( 'NONE',  ( -6.700000000000019718, 12.50000000000000000, -2.385244779468109755E-15 ) ) ;
#121588=ORIENTED_EDGE ( 'NONE', *, *, #73218, .T. ) ;
#121589=ORIENTED_EDGE ( 'NONE', *, *, #58558, .T. ) ;
#121590=ORIENTED_EDGE ( 'NONE', *, *, #86630, .T. ) ;
#121592=CIRCLE ( 'NONE', #46287, 0.06509327318403745899 ) ;
#121593=ORIENTED_EDGE ( 'NONE', *, *, #61057, .F. ) ;
#121594=DIRECTION ( 'NONE',  ( -0.000000000000000000, 1.000000000000000000, -0.000000000000000000 ) ) ;
#121595=LINE ( 'NONE', #83629, #56119 ) ;
#121596=AXIS2_PLACEMENT_3D ( 'NONE', #63029, #62397, #1519 ) ;
#121597=LINE ( 'NONE', #101336, #111747 ) ;
#121598=CARTESIAN_POINT ( 'NONE',  ( 8.549999999999924327, 2.500000000000000000, -6.841600689897077814 ) ) ;
#121599=CARTESIAN_POINT ( 'NONE',  ( 12.49999999999990408, 2.500000000000000000, 5.122947341949749323 ) ) ;
#121600=DIRECTION ( 'NONE',  ( -0.000000000000000000, -1.000000000000000000, -0.000000000000000000 ) ) ;
#121601=DIRECTION ( 'NONE',  ( 0.000000000000000000, 0.000000000000000000, 1.000000000000000000 ) ) ;
#121602=DIRECTION ( 'NONE',  ( 0.000000000000000000, 1.000000000000000000, 0.000000000000000000 ) ) ;
#121603=AXIS2_PLACEMENT_3D ( 'NONE', #70640, #28145, #30096 ) ;
#121604=ORIENTED_EDGE ( 'NONE', *, *, #30070, .T. ) ;
#121605=CIRCLE ( 'NONE', #25445, 0.1000000000000000472 ) ;
#121606=AXIS2_PLACEMENT_3D ( 'NONE', #54868, #76462, #124914 ) ;
#121607=LINE ( 'NONE', #72534, #2649 ) ;
#121608=CONICAL_SURFACE ( 'NONE', #56744, 0.1000000000000002554, 0.003490658503988666988 ) ;
#121609=CARTESIAN_POINT ( 'NONE',  ( -4.800000000000022915, 2.500000000000000000, -0.2464101615137783419 ) ) ;
#121610=ORIENTED_EDGE ( 'NONE', *, *, #76568, .T. ) ;
#121611=EDGE_LOOP ( 'NONE', ( #67142, #76017 ) ) ;
#121613=CARTESIAN_POINT ( 'NONE',  ( -8.550000000000013145, 2.500000000000000000, -6.941600689897073906 ) ) ;
#121614=DIRECTION ( 'NONE',  ( -0.000000000000000000, 1.000000000000000000, -0.000000000000000000 ) ) ;
#121615=VECTOR ( 'NONE', #125379, 1000.000000000000000 ) ;
#121616=LINE ( 'NONE', #62725, #55220 ) ;
#121617=CARTESIAN_POINT ( 'NONE',  ( 3.349999999999945466, 12.50000000000000000, -7.253104124594891289 ) ) ;
#121618=AXIS2_PLACEMENT_3D ( 'NONE', #61823, #32382, #22547 ) ;
#121619=ADVANCED_FACE ( 'NONE', ( #91675 ), #110903, .T. ) ;
#121620=CARTESIAN_POINT ( 'NONE',  ( -6.700000000000019718, 12.50000000000000000, -2.385244779468109755E-15 ) ) ;
#121621=CIRCLE ( 'NONE', #6669, 0.1000000000000000056 ) ;
#121622=DIRECTION ( 'NONE',  ( 0.000000000000000000, -0.9999939076577903929, 0.003490651415223739937 ) ) ;
#121623=VECTOR ( 'NONE', #21813, 1000.000000000000000 ) ;
#121624=DIRECTION ( 'NONE',  ( 0.000000000000000000, 0.000000000000000000, 1.000000000000000000 ) ) ;
#121625=AXIS2_PLACEMENT_3D ( 'NONE', #38362, #86128, #17392 ) ;
#121626=AXIS2_PLACEMENT_3D ( 'NONE', #122026, #289, #61827 ) ;
#121627=LINE ( 'NONE', #90223, #85546 ) ;
#121628=EDGE_CURVE ( 'NONE', #84054, #111888, #29450, .T. ) ;
#121630=ORIENTED_EDGE ( 'NONE', *, *, #103821, .F. ) ;
#121631=AXIS2_PLACEMENT_3D ( 'NONE', #96262, #54415, #74709 ) ;
#121632=ORIENTED_EDGE ( 'NONE', *, *, #16067, .T. ) ;
#121633=EDGE_CURVE ( 'NONE', #50907, #14841, #83815, .T. ) ;
#121634=VERTEX_POINT ( 'NONE', #33418 ) ;
#121635=EDGE_CURVE ( 'NONE', #92388, #89740, #60840, .T. ) ;
#121636=CARTESIAN_POINT ( 'NONE',  ( -1.250000000000037970, 12.50000000000000000, 7.188010851410848723 ) ) ;
#121637=CARTESIAN_POINT ( 'NONE',  ( 5.199999999999933564, 12.50000000000000000, 3.983716857408420076 ) ) ;
#121638=ORIENTED_EDGE ( 'NONE', *, *, #75222, .T. ) ;
#121639=CARTESIAN_POINT ( 'NONE',  ( -2.900000000000029221, 2.500000000000000000, -4.330127018922201643 ) ) ;
#121640=DIRECTION ( 'NONE',  ( 0.000000000000000000, 0.000000000000000000, -1.000000000000000000 ) ) ;
#121641=EDGE_CURVE ( 'NONE', #46605, #125318, #69144, .T. ) ;
#121642=DIRECTION ( 'NONE',  ( 0.000000000000000000, 0.000000000000000000, 1.000000000000000000 ) ) ;
#121643=DIRECTION ( 'NONE',  ( 0.000000000000000000, 0.000000000000000000, 1.000000000000000000 ) ) ;
#121644=VERTEX_POINT ( 'NONE', #121767 ) ;
#121645=ADVANCED_FACE ( 'NONE', ( #11817 ), #14834, .T. ) ;
#121646=CARTESIAN_POINT ( 'NONE',  ( -4.550000000000026468, 2.500000000000000000, -6.395190528383301931 ) ) ;
#121647=DIRECTION ( 'NONE',  ( 0.000000000000000000, -0.000000000000000000, 1.000000000000000000 ) ) ;
#121648=VERTEX_POINT ( 'NONE', #73310 ) ;
#121649=ORIENTED_EDGE ( 'NONE', *, *, #80724, .T. ) ;
#121650=ORIENTED_EDGE ( 'NONE', *, *, #109737, .F. ) ;
#121651=AXIS2_PLACEMENT_3D ( 'NONE', #99974, #59426, #99331 ) ;
#121652=ORIENTED_EDGE ( 'NONE', *, *, #109832, .F. ) ;
#121653=CARTESIAN_POINT ( 'NONE',  ( -10.20000000000000462, 2.500000000000000000, 0.2464101615137735679 ) ) ;
#121654=CONICAL_SURFACE ( 'NONE', #88279, 0.1000000000000000472, 0.003490658503988666988 ) ;
#121655=VECTOR ( 'NONE', #18429, 1000.000000000000000 ) ;
#121656=DIRECTION ( 'NONE',  ( -0.000000000000000000, -1.000000000000000000, -0.000000000000000000 ) ) ;
#121657=CARTESIAN_POINT ( 'NONE',  ( -11.44999999999999751, 12.50000000000000000, -6.841600689897074261 ) ) ;
#121658=AXIS2_PLACEMENT_3D ( 'NONE', #13323, #53280, #83996 ) ;
#121659=EDGE_LOOP ( 'NONE', ( #69175, #47331, #60244, #46203 ) ) ;
#121660=AXIS2_PLACEMENT_3D ( 'NONE', #102167, #52412, #92331 ) ;
#121661=AXIS2_PLACEMENT_3D ( 'NONE', #33697, #4217, #16449 ) ;
#121662=CARTESIAN_POINT ( 'NONE',  ( 3.349999999999945466, 12.50000000000000000, -6.495190528383302464 ) ) ;
#121664=FACE_OUTER_BOUND ( 'NONE', #49060, .T. ) ;
#121665=CARTESIAN_POINT ( 'NONE',  ( 16.70850060796060887, -0.4765610498145435026, -5.930927070179899729 ) ) ;
#121666=AXIS2_PLACEMENT_3D ( 'NONE', #82055, #61796, #32352 ) ;
#121667=DIRECTION ( 'NONE',  ( 0.000000000000000000, 0.000000000000000000, 1.000000000000000000 ) ) ;
#121668=DIRECTION ( 'NONE',  ( -0.000000000000000000, 1.000000000000000000, -0.000000000000000000 ) ) ;
#121669=CIRCLE ( 'NONE', #61135, 0.06509327318403745899 ) ;
#121670=VERTEX_POINT ( 'NONE', #51758 ) ;
#121671=VERTEX_POINT ( 'NONE', #102145 ) ;
#121672=ORIENTED_EDGE ( 'NONE', *, *, #11133, .T. ) ;
#121673=CARTESIAN_POINT ( 'NONE',  ( -2.050000000000033129, 12.50000000000000000, 2.165063509461097713 ) ) ;
#121674=DIRECTION ( 'NONE',  ( 0.000000000000000000, 0.000000000000000000, -1.000000000000000000 ) ) ;
#121675=DIRECTION ( 'NONE',  ( -4.274815082592931898E-19, -0.9999939076577903929, -0.003490651415223739937 ) ) ;
#121676=FACE_BOUND ( 'NONE', #80215, .T. ) ;
#121677=DIRECTION ( 'NONE',  ( -4.274815082592931898E-19, -0.9999939076577903929, -0.003490651415223739937 ) ) ;
#121678=FACE_OUTER_BOUND ( 'NONE', #97780, .T. ) ;
#121679=EDGE_CURVE ( 'NONE', #75247, #104608, #6417, .T. ) ;
#121680=DIRECTION ( 'NONE',  ( 0.000000000000000000, 1.000000000000000000, 0.000000000000000000 ) ) ;
#121681=ADVANCED_FACE ( 'NONE', ( #23574 ), #98467, .T. ) ;
#121682=ADVANCED_FACE ( 'NONE', ( #72686 ), #94277, .T. ) ;
#121683=DIRECTION ( 'NONE',  ( 0.000000000000000000, 1.000000000000000000, 0.000000000000000000 ) ) ;
#121684=DIRECTION ( 'NONE',  ( -0.000000000000000000, 1.000000000000000000, -0.000000000000000000 ) ) ;
#121685=ADVANCED_FACE ( 'NONE', ( #41944 ), #104731, .T. ) ;
#121686=DIRECTION ( 'NONE',  ( 0.000000000000000000, 0.000000000000000000, 1.000000000000000000 ) ) ;
#121687=EDGE_LOOP ( 'NONE', ( #30122, #129229 ) ) ;
#121688=EDGE_CURVE ( 'NONE', #73789, #83814, #121465, .T. ) ;
#121689=CARTESIAN_POINT ( 'NONE',  ( -1.850000000000033396, 12.50000000000000000, -2.446380397790840266 ) ) ;
#121690=CARTESIAN_POINT ( 'NONE',  ( -8.750000000000007105, 2.500000000000000000, 7.088010851410848190 ) ) ;
#121691=ADVANCED_FACE ( 'NONE', ( #73968 ), #21212, .T. ) ;
#121692=EDGE_LOOP ( 'NONE', ( #37473, #124734, #8099, #80983 ) ) ;
#121693=EDGE_LOOP ( 'NONE', ( #76999, #100752 ) ) ;
#121694=DIRECTION ( 'NONE',  ( 0.000000000000000000, 0.000000000000000000, -1.000000000000000000 ) ) ;
#121695=DIRECTION ( 'NONE',  ( 0.000000000000000000, 1.000000000000000000, 0.000000000000000000 ) ) ;
#121696=FACE_BOUND ( 'NONE', #116148, .T. ) ;
#121697=AXIS2_PLACEMENT_3D ( 'NONE', #88164, #27319, #109101 ) ;
#121698=CARTESIAN_POINT ( 'NONE',  ( 7.049999999999930544, 2.500000000000000000, -6.495190528383302464 ) ) ;
#121699=CIRCLE ( 'NONE', #65254, 0.06509327318403745899 ) ;
#121700=EDGE_CURVE ( 'NONE', #68510, #68006, #65012, .T. ) ;
#121701=AXIS2_PLACEMENT_3D ( 'NONE', #109396, #120516, #89118 ) ;
#121702=EDGE_CURVE ( 'NONE', #6433, #73886, #113155, .T. ) ;
#121703=ORIENTED_EDGE ( 'NONE', *, *, #96260, .F. ) ;
#121704=CARTESIAN_POINT ( 'NONE',  ( 10.64999999999991331, 2.500000000000000000, 6.941600689897073018 ) ) ;
#121705=CARTESIAN_POINT ( 'NONE',  ( 11.44999999999990870, 2.500000000000000000, -1.818653347947326138 ) ) ;
#121706=VERTEX_POINT ( 'NONE', #102766 ) ;
#121707=CIRCLE ( 'NONE', #102932, 0.1000000000000000472 ) ;
#121708=PLANE ( 'NONE',  #38621 ) ;
#121709=DIRECTION ( 'NONE',  ( 0.000000000000000000, -0.000000000000000000, 1.000000000000000000 ) ) ;
#121710=VECTOR ( 'NONE', #120575, 1000.000000000000000 ) ;
#121711=AXIS2_PLACEMENT_3D ( 'NONE', #91022, #58986, #81208 ) ;
#121712=CONICAL_SURFACE ( 'NONE', #102940, 0.1000000000000002554, 0.003490658503988666988 ) ;
#121713=CIRCLE ( 'NONE', #104978, 0.06509327318403745899 ) ;
#121714=VERTEX_POINT ( 'NONE', #53046 ) ;
#121715=DIRECTION ( 'NONE',  ( -0.000000000000000000, -1.000000000000000000, -0.000000000000000000 ) ) ;
#121716=CARTESIAN_POINT ( 'NONE',  ( -2.700000000000030820, 2.500000000000000000, -3.883716857408426648 ) ) ;
#121717=AXIS2_PLACEMENT_3D ( 'NONE', #34638, #121695, #84358 ) ;
#121718=ORIENTED_EDGE ( 'NONE', *, *, #120361, .F. ) ;
#121719=DIRECTION ( 'NONE',  ( -0.000000000000000000, -1.000000000000000000, -0.000000000000000000 ) ) ;
#121720=AXIS2_PLACEMENT_3D ( 'NONE', #29481, #109321, #118489 ) ;
#121721=DIRECTION ( 'NONE',  ( -0.000000000000000000, -1.000000000000000000, -0.000000000000000000 ) ) ;
#121722=CARTESIAN_POINT ( 'NONE',  ( -5.000000000000023093, 12.50000000000000000, 0.6277270498435120194 ) ) ;
#121723=VERTEX_POINT ( 'NONE', #92975 ) ;
#121724=ORIENTED_EDGE ( 'NONE', *, *, #101862, .F. ) ;
#121725=CARTESIAN_POINT ( 'NONE',  ( -9.400000000000007461, 12.50000000000000000, 0.3464101615137735735 ) ) ;
#121726=EDGE_LOOP ( 'NONE', ( #75609, #84724, #112586, #15640 ) ) ;
#121727=FACE_OUTER_BOUND ( 'NONE', #63529, .T. ) ;
#121728=CARTESIAN_POINT ( 'NONE',  ( 15.19999999999989271, 2.500000000000000000, -0.4464101615137783252 ) ) ;
#121729=CARTESIAN_POINT ( 'NONE',  ( -13.54999999999999005, 2.500000000000000000, 2.511473670974877503 ) ) ;
#121730=EDGE_LOOP ( 'NONE', ( #10748, #75751, #4489, #59091 ) ) ;
#121731=FACE_OUTER_BOUND ( 'NONE', #78820, .T. ) ;
#121732=DIRECTION ( 'NONE',  ( -0.000000000000000000, 1.000000000000000000, -0.000000000000000000 ) ) ;
#121733=DIRECTION ( 'NONE',  ( 0.000000000000000000, 0.000000000000000000, 1.000000000000000000 ) ) ;
#121734=DIRECTION ( 'NONE',  ( 0.000000000000000000, -0.9999939076577903929, 0.003490651415223739937 ) ) ;
#121735=FACE_OUTER_BOUND ( 'NONE', #15733, .T. ) ;
#121736=DIRECTION ( 'NONE',  ( -0.000000000000000000, 1.000000000000000000, -0.000000000000000000 ) ) ;
#121737=ORIENTED_EDGE ( 'NONE', *, *, #57893, .T. ) ;
#121738=ADVANCED_FACE ( 'NONE', ( #3297 ), #74612, .T. ) ;
#121740=DIRECTION ( 'NONE',  ( -0.000000000000000000, 1.000000000000000000, -0.000000000000000000 ) ) ;
#121741=ORIENTED_EDGE ( 'NONE', *, *, #126281, .F. ) ;
#121742=AXIS2_PLACEMENT_3D ( 'NONE', #60558, #9502, #38995 ) ;
#121743=CARTESIAN_POINT ( 'NONE',  ( 11.69999999999990514, 12.50000000000000000, -2.276824562219559311E-15 ) ) ;
#121744=AXIS2_PLACEMENT_3D ( 'NONE', #52355, #62829, #92270 ) ;
#121745=CIRCLE ( 'NONE', #6794, 0.06509327318403745899 ) ;
#121746=ORIENTED_EDGE ( 'NONE', *, *, #115979, .T. ) ;
#121747=ORIENTED_EDGE ( 'NONE', *, *, #118278, .T. ) ;
#121748=VERTEX_POINT ( 'NONE', #55615 ) ;
#121749=DIRECTION ( 'NONE',  ( 0.000000000000000000, 0.000000000000000000, -1.000000000000000000 ) ) ;
#121750=LINE ( 'NONE', #72031, #4650 ) ;
#121751=AXIS2_PLACEMENT_3D ( 'NONE', #115147, #35979, #64784 ) ;
#121752=AXIS2_PLACEMENT_3D ( 'NONE', #118420, #30062, #58864 ) ;
#121753=FACE_OUTER_BOUND ( 'NONE', #85183, .T. ) ;
#121754=AXIS2_PLACEMENT_3D ( 'NONE', #101485, #41925, #83141 ) ;
#121755=LINE ( 'NONE', #14999, #32728 ) ;
#121756=DIRECTION ( 'NONE',  ( -0.000000000000000000, 1.000000000000000000, -0.000000000000000000 ) ) ;
#121757=LINE ( 'NONE', #72035, #119657 ) ;
#121758=AXIS2_PLACEMENT_3D ( 'NONE', #6442, #46393, #86314 ) ;
#121759=CARTESIAN_POINT ( 'NONE',  ( 1.649999999999948841, 2.500000000000000000, 6.595190528383296780 ) ) ;
#121760=CARTESIAN_POINT ( 'NONE',  ( 6.449999999999930012, 12.50000000000000000, 6.906693963081109722 ) ) ;
#121761=CARTESIAN_POINT ( 'NONE',  ( 0.3999999999999555023, 2.500000000000000000, 4.330127018922196314 ) ) ;
#121762=CIRCLE ( 'NONE', #111373, 0.1000000000000000056 ) ;
#121763=ORIENTED_EDGE ( 'NONE', *, *, #22406, .F. ) ;
#121764=CARTESIAN_POINT ( 'NONE',  ( 14.79999999999989235, 12.50000000000000000, 0.3464101615137735735 ) ) ;
#121765=ORIENTED_EDGE ( 'NONE', *, *, #29572, .F. ) ;
#121766=ORIENTED_EDGE ( 'NONE', *, *, #57166, .F. ) ;
#121767=CARTESIAN_POINT ( 'NONE',  ( 12.89999999999990266, 12.50000000000000000, -5.088040615133791356 ) ) ;
#121768=LINE ( 'NONE', #51759, #20452 ) ;
#121769=CARTESIAN_POINT ( 'NONE',  ( 11.44999999999990870, 12.50000000000000000, 6.841600689897072485 ) ) ;
#121770=CARTESIAN_POINT ( 'NONE',  ( -11.64999999999999680, 2.500000000000000000, 2.165063509461097713 ) ) ;
#121771=DIRECTION ( 'NONE',  ( 0.000000000000000000, 0.000000000000000000, 1.000000000000000000 ) ) ;
#121772=DIRECTION ( 'NONE',  ( -0.000000000000000000, 1.000000000000000000, -0.000000000000000000 ) ) ;
#121773=CARTESIAN_POINT ( 'NONE',  ( 5.649999999999936406, 12.50000000000000000, -6.083687093685488989 ) ) ;
#121774=EDGE_LOOP ( 'NONE', ( #47223, #124503, #46843, #87196 ) ) ;
#121775=EDGE_LOOP ( 'NONE', ( #37182, #63716, #84334, #35801 ) ) ;
#121776=ADVANCED_FACE ( 'NONE', ( #114520 ), #110992, .T. ) ;
#121777=VECTOR ( 'NONE', #86455, 1000.000000000000000 ) ;
#121778=ORIENTED_EDGE ( 'NONE', *, *, #110865, .F. ) ;
#121779=ORIENTED_EDGE ( 'NONE', *, *, #21327, .T. ) ;
#121780=ADVANCED_FACE ( 'NONE', ( #116457 ), #42068, .T. ) ;
#121781=ORIENTED_EDGE ( 'NONE', *, *, #32172, .T. ) ;
#121782=CIRCLE ( 'NONE', #90382, 0.1000000000000002554 ) ;
#121783=EDGE_CURVE ( 'NONE', #92818, #56590, #54556, .T. ) ;
#121785=DIRECTION ( 'NONE',  ( -0.000000000000000000, -1.000000000000000000, -0.000000000000000000 ) ) ;
#121786=AXIS2_PLACEMENT_3D ( 'NONE', #31964, #81062, #112458 ) ;
#121787=AXIS2_PLACEMENT_3D ( 'NONE', #102266, #73429, #103559 ) ;
#121788=CARTESIAN_POINT ( 'NONE',  ( 12.49999999999993960, 12.50000000000000000, 4.330127018922196314 ) ) ;
#121789=AXIS2_PLACEMENT_3D ( 'NONE', #40867, #110849, #61120 ) ;
#121790=DIRECTION ( 'NONE',  ( 0.000000000000000000, 1.000000000000000000, 0.000000000000000000 ) ) ;
#121791=ADVANCED_FACE ( 'NONE', ( #115820 ), #85710, .T. ) ;
#121792=DIRECTION ( 'NONE',  ( 0.000000000000000000, 0.000000000000000000, 1.000000000000000000 ) ) ;
#121793=EDGE_CURVE ( 'NONE', #56841, #35476, #25312, .T. ) ;
#121794=ORIENTED_EDGE ( 'NONE', *, *, #71246, .T. ) ;
#121795=CARTESIAN_POINT ( 'NONE',  ( 0.3999999999999628852, 2.500000000000000000, -0.7928203230275520097 ) ) ;
#121796=CARTESIAN_POINT ( 'NONE',  ( -10.45000000000000462, 2.500000000000000000, -2.165063509461097713 ) ) ;
#121797=EDGE_CURVE ( 'NONE', #110118, #22205, #37845, .T. ) ;
#121798=FACE_OUTER_BOUND ( 'NONE', #53785, .T. ) ;
#121799=EDGE_CURVE ( 'NONE', #108367, #106850, #26802, .T. ) ;
#121800=LINE ( 'NONE', #3325, #32632 ) ;
#121801=AXIS2_PLACEMENT_3D ( 'NONE', #128300, #118455, #50367 ) ;
#121802=AXIS2_PLACEMENT_3D ( 'NONE', #65512, #17694, #88359 ) ;
#121803=DIRECTION ( 'NONE',  ( -0.000000000000000000, 1.000000000000000000, -0.000000000000000000 ) ) ;
#121804=ORIENTED_EDGE ( 'NONE', *, *, #108817, .F. ) ;
#121805=AXIS2_PLACEMENT_3D ( 'NONE', #49673, #100045, #58201 ) ;
#121806=AXIS2_PLACEMENT_3D ( 'NONE', #32780, #45802, #13736 ) ;
#121807=EDGE_LOOP ( 'NONE', ( #6018, #20355 ) ) ;
#121808=ORIENTED_EDGE ( 'NONE', *, *, #74940, .T. ) ;
#121809=FACE_OUTER_BOUND ( 'NONE', #120288, .T. ) ;
#121810=EDGE_CURVE ( 'NONE', #75902, #84566, #127735, .T. ) ;
#121811=CIRCLE ( 'NONE', #82109, 0.09999999999999999167 ) ;
#121812=VERTEX_POINT ( 'NONE', #37279 ) ;
#121813=FACE_OUTER_BOUND ( 'NONE', #6691, .T. ) ;
#121814=FACE_OUTER_BOUND ( 'NONE', #75867, .T. ) ;
#121815=CIRCLE ( 'NONE', #117587, 0.1000000000000002554 ) ;
#121816=EDGE_LOOP ( 'NONE', ( #47891, #101651 ) ) ;
#121817=CARTESIAN_POINT ( 'NONE',  ( -8.750000000000005329, 2.500000000000000000, 5.702370205355745014 ) ) ;
#121818=CARTESIAN_POINT ( 'NONE',  ( -12.49999999999999289, 12.50000000000000000, 3.702399969078682407 ) ) ;
#121819=CARTESIAN_POINT ( 'NONE',  ( -14.54999999999998472, 2.500000000000000000, -2.065063509461099844 ) ) ;
#121820=CARTESIAN_POINT ( 'NONE',  ( 4.349999999999941025, 2.500000000000000000, -6.148780366869526226 ) ) ;
#121821=CARTESIAN_POINT ( 'NONE',  ( 7.699999999999923794, 12.50000000000000000, -0.3464101615137783474 ) ) ;
#121822=ORIENTED_EDGE ( 'NONE', *, *, #117835, .T. ) ;
#121823=AXIS2_PLACEMENT_3D ( 'NONE', #70099, #58990, #98900 ) ;
#121825=CONICAL_SURFACE ( 'NONE', #52888, 0.09999999999999999167, 0.003490658503988666988 ) ;
#121826=EDGE_CURVE ( 'NONE', #93625, #97708, #71288, .T. ) ;
#121827=CARTESIAN_POINT ( 'NONE',  ( 7.899999999999924860, 2.500000000000000000, -3.537306695894649966 ) ) ;
#121828=DIRECTION ( 'NONE',  ( 0.000000000000000000, -0.9999939076577903929, 0.003490651415223739937 ) ) ;
#121829=DIRECTION ( 'NONE',  ( 0.000000000000000000, 0.000000000000000000, 1.000000000000000000 ) ) ;
#121830=LINE ( 'NONE', #12519, #41730 ) ;
#121832=CONICAL_SURFACE ( 'NONE', #109318, 0.1000000000000002554, 0.003490658503988666988 ) ;
#121833=AXIS2_PLACEMENT_3D ( 'NONE', #28431, #19904, #59849 ) ;
#121834=VERTEX_POINT ( 'NONE', #97472 ) ;
#121835=EDGE_CURVE ( 'NONE', #24133, #99929, #92216, .T. ) ;
#121836=DIRECTION ( 'NONE',  ( -4.274815082592931898E-19, -0.9999939076577903929, -0.003490651415223739937 ) ) ;
#121837=DIRECTION ( 'NONE',  ( -0.000000000000000000, -1.000000000000000000, -0.000000000000000000 ) ) ;
#121838=DIRECTION ( 'NONE',  ( -0.000000000000000000, -1.000000000000000000, -0.000000000000000000 ) ) ;
#121839=ADVANCED_FACE ( 'NONE', ( #126295 ), #47739, .T. ) ;
#121840=CARTESIAN_POINT ( 'NONE',  ( -7.300000000000016698, 12.50000000000000000, -4.611443907251940644 ) ) ;
#121841=ORIENTED_EDGE ( 'NONE', *, *, #73987, .T. ) ;
#121842=CIRCLE ( 'NONE', #4754, 0.09999999999999982514 ) ;
#121843=CARTESIAN_POINT ( 'NONE',  ( 8.749999999999923617, 12.50000000000000000, 1.407149913249508000 ) ) ;
#121844=CIRCLE ( 'NONE', #126041, 0.06509327318403745899 ) ;
#121845=EDGE_CURVE ( 'NONE', #79920, #8444, #35798, .T. ) ;
#121846=DIRECTION ( 'NONE',  ( 0.000000000000000000, 0.000000000000000000, 1.000000000000000000 ) ) ;
#121847=CIRCLE ( 'NONE', #11025, 0.09999999999999982514 ) ;
#121848=VERTEX_POINT ( 'NONE', #47101 ) ;
#121849=CIRCLE ( 'NONE', #52910, 0.1000000000000002554 ) ;
#121850=DIRECTION ( 'NONE',  ( 0.000000000000000000, 1.000000000000000000, 0.000000000000000000 ) ) ;
#121851=EDGE_CURVE ( 'NONE', #7001, #55449, #52521, .T. ) ;
#121852=ORIENTED_EDGE ( 'NONE', *, *, #41722, .T. ) ;
#121853=CIRCLE ( 'NONE', #88388, 0.1000000000000002554 ) ;
#121854=CARTESIAN_POINT ( 'NONE',  ( 1.049999999999954081, 12.50000000000000000, -6.213873640053564351 ) ) ;
#121855=EDGE_CURVE ( 'NONE', #35899, #30305, #85947, .T. ) ;
#121856=ADVANCED_FACE ( 'NONE', ( #124999 ), #123608, .T. ) ;
#121857=ADVANCED_FACE ( 'NONE', ( #117092 ), #29541, .T. ) ;
#121858=EDGE_LOOP ( 'NONE', ( #63137, #84935 ) ) ;
#121859=DIRECTION ( 'NONE',  ( 0.000000000000000000, 0.000000000000000000, 1.000000000000000000 ) ) ;
#121860=CARTESIAN_POINT ( 'NONE',  ( 12.30568799055497564, 2.500000000000001776, -7.490555763477717122 ) ) ;
#121861=VERTEX_POINT ( 'NONE', #49686 ) ;
#121862=ORIENTED_EDGE ( 'NONE', *, *, #25800, .T. ) ;
#121863=CARTESIAN_POINT ( 'NONE',  ( -7.300000000000013145, 2.500000000000000000, 4.083716857408420609 ) ) ;
#121864=CARTESIAN_POINT ( 'NONE',  ( -3.750000000000031086, 2.500000000000000000, -5.902370205355750521 ) ) ;
#121865=EDGE_CURVE ( 'NONE', #68456, #45964, #6510, .T. ) ;
#121866=AXIS2_PLACEMENT_3D ( 'NONE', #121195, #31535, #119913 ) ;
#121867=LINE ( 'NONE', #1444, #80280 ) ;
#121869=DIRECTION ( 'NONE',  ( 0.000000000000000000, -0.9999939076577903929, 0.003490651415223739937 ) ) ;
#121870=CARTESIAN_POINT ( 'NONE',  ( -14.79999999999998472, 2.500000000000000000, 0.3464101615137758494 ) ) ;
#121871=CARTESIAN_POINT ( 'NONE',  ( -3.750000000000031086, 2.500000000000000000, -5.702370205355749455 ) ) ;
#121872=DIRECTION ( 'NONE',  ( 0.000000000000000000, 0.000000000000000000, 1.000000000000000000 ) ) ;
#121873=CARTESIAN_POINT ( 'NONE',  ( 1.649999999999951505, 2.500000000000000000, -2.857883832488653741 ) ) ;
#121874=CIRCLE ( 'NONE', #27778, 0.06509327318403745899 ) ;
#121875=CIRCLE ( 'NONE', #80119, 0.1000000000000000472 ) ;
#121876=CIRCLE ( 'NONE', #86368, 0.09999999999999982514 ) ;
#121877=VERTEX_POINT ( 'NONE', #39868 ) ;
#121878=ORIENTED_EDGE ( 'NONE', *, *, #62147, .F. ) ;
#121879=DIRECTION ( 'NONE',  ( 0.000000000000000000, 0.000000000000000000, 1.000000000000000000 ) ) ;
#121880=EDGE_LOOP ( 'NONE', ( #36752, #40044, #72942, #38879 ) ) ;
#121881=CARTESIAN_POINT ( 'NONE',  ( 12.69999999999989981, 12.50000000000000000, -0.4115034346978157509 ) ) ;
#121882=CARTESIAN_POINT ( 'NONE',  ( -2.900000000000030109, 12.50000000000000000, -3.637306695894650055 ) ) ;
#121883=DIRECTION ( 'NONE',  ( 0.000000000000000000, 0.000000000000000000, 1.000000000000000000 ) ) ;
#121884=EDGE_LOOP ( 'NONE', ( #41651, #30416, #60862, #67098 ) ) ;
#121885=EDGE_LOOP ( 'NONE', ( #68610, #66011 ) ) ;
#121886=FACE_BOUND ( 'NONE', #24674, .T. ) ;
#121887=ORIENTED_EDGE ( 'NONE', *, *, #15974, .F. ) ;
#121888=CIRCLE ( 'NONE', #98901, 0.1000000000000002554 ) ;
#121889=DIRECTION ( 'NONE',  ( -0.000000000000000000, -1.000000000000000000, -0.000000000000000000 ) ) ;
#121890=DIRECTION ( 'NONE',  ( 0.000000000000000000, 1.000000000000000000, 0.000000000000000000 ) ) ;
#121891=VECTOR ( 'NONE', #45003, 1000.000000000000000 ) ;
#121892=AXIS2_PLACEMENT_3D ( 'NONE', #42722, #94359, #91795 ) ;
#121893=LINE ( 'NONE', #123194, #61786 ) ;
#121894=CARTESIAN_POINT ( 'NONE',  ( 6.249999999999968914, 12.50000000000000000, -6.495190528383302464 ) ) ;
#121895=AXIS2_PLACEMENT_3D ( 'NONE', #32817, #103471, #104117 ) ;
#121896=DIRECTION ( 'NONE',  ( -4.274815082592931898E-19, -0.9999939076577903929, -0.003490651415223739937 ) ) ;
#121897=DIRECTION ( 'NONE',  ( -0.000000000000000000, 1.000000000000000000, -0.000000000000000000 ) ) ;
#121898=DIRECTION ( 'NONE',  ( 0.000000000000000000, 0.000000000000000000, 1.000000000000000000 ) ) ;
#121899=DIRECTION ( 'NONE',  ( 0.000000000000000000, -0.000000000000000000, 1.000000000000000000 ) ) ;
#121900=CARTESIAN_POINT ( 'NONE',  ( -8.950000000000009948, 2.500000000000000000, -6.741600689897071952 ) ) ;
#121901=CARTESIAN_POINT ( 'NONE',  ( -11.89999999999999680, 2.500000000000000000, -0.3464101615137741841 ) ) ;
#121902=CIRCLE ( 'NONE', #61275, 0.06509327318403745899 ) ;
#121903=DIRECTION ( 'NONE',  ( 0.000000000000000000, 0.000000000000000000, 1.000000000000000000 ) ) ;
#121904=EDGE_LOOP ( 'NONE', ( #49280, #124448 ) ) ;
#121905=ORIENTED_EDGE ( 'NONE', *, *, #118116, .F. ) ;
#121907=ORIENTED_EDGE ( 'NONE', *, *, #129287, .T. ) ;
#121908=DIRECTION ( 'NONE',  ( -0.000000000000000000, -1.000000000000000000, -0.000000000000000000 ) ) ;
#121909=AXIS2_PLACEMENT_3D ( 'NONE', #108963, #118160, #90633 ) ;
#121910=EDGE_LOOP ( 'NONE', ( #57705, #96133 ) ) ;
#121911=VECTOR ( 'NONE', #8123, 1000.000000000000000 ) ;
#121912=AXIS2_PLACEMENT_3D ( 'NONE', #90841, #81029, #120941 ) ;
#121913=DIRECTION ( 'NONE',  ( 0.000000000000000000, 0.000000000000000000, 1.000000000000000000 ) ) ;
#121914=CARTESIAN_POINT ( 'NONE',  ( -3.550000000000027800, 2.500000000000000000, 6.048780366869520364 ) ) ;
#121915=ORIENTED_EDGE ( 'NONE', *, *, #75545, .T. ) ;
#121916=EDGE_LOOP ( 'NONE', ( #84452, #113055 ) ) ;
#121917=EDGE_LOOP ( 'NONE', ( #10616, #64290, #96168, #7398 ) ) ;
#121918=CONICAL_SURFACE ( 'NONE', #25761, 0.1000000000000002554, 0.003490658503988666988 ) ;
#121919=CARTESIAN_POINT ( 'NONE',  ( 7.699999999999922018, 2.500000000000000000, 0.3464101615137735735 ) ) ;
#121920=CARTESIAN_POINT ( 'NONE',  ( -10.20000000000000462, 12.50000000000000000, 0.3464101615137735735 ) ) ;
#121921=CONICAL_SURFACE ( 'NONE', #12950, 0.1000000000000002554, 0.003490658503988666988 ) ;
#121922=( NAMED_UNIT ( * ) SI_UNIT ( $, .STERADIAN. ) SOLID_ANGLE_UNIT ( ) );
#121923=CARTESIAN_POINT ( 'NONE',  ( 2.499999999999947153, 2.500000000000000000, 3.737306695894644371 ) ) ;
#121924=CARTESIAN_POINT ( 'NONE',  ( 8.149999999999923972, 12.50000000000000000, -6.213873640053564351 ) ) ;
#121925=DIRECTION ( 'NONE',  ( -0.000000000000000000, -1.000000000000000000, -0.000000000000000000 ) ) ;
#121926=DIRECTION ( 'NONE',  ( 0.000000000000000000, 0.000000000000000000, 1.000000000000000000 ) ) ;
#121927=EDGE_CURVE ( 'NONE', #14735, #72399, #104560, .T. ) ;
#121928=VERTEX_POINT ( 'NONE', #106495 ) ;
#121929=CARTESIAN_POINT ( 'NONE',  ( -6.650000000000015454, 2.500000000000000000, 7.188010851410848723 ) ) ;
#121930=ORIENTED_EDGE ( 'NONE', *, *, #7406, .T. ) ;
#121931=ORIENTED_EDGE ( 'NONE', *, *, #56952, .F. ) ;
#121932=VERTEX_POINT ( 'NONE', #124204 ) ;
#121933=CARTESIAN_POINT ( 'NONE',  ( -3.469446951953614189E-14, 2.500000000000000000, -0.6928203230275519209 ) ) ;
#121934=CIRCLE ( 'NONE', #55126, 0.06509327318403745899 ) ;
#121935=VECTOR ( 'NONE', #42547, 1000.000000000000000 ) ;
#121936=VERTEX_POINT ( 'NONE', #85561 ) ;
#121937=ORIENTED_EDGE ( 'NONE', *, *, #114871, .F. ) ;
#121938=ORIENTED_EDGE ( 'NONE', *, *, #65545, .T. ) ;
#121940=AXIS2_PLACEMENT_3D ( 'NONE', #76916, #16040, #57933 ) ;
#121941=CARTESIAN_POINT ( 'NONE',  ( 9.349999999999919709, 12.50000000000000000, 1.818653347947321475 ) ) ;
#121942=CARTESIAN_POINT ( 'NONE',  ( -8.950000000000006395, 12.50000000000000000, 6.906693963081109722 ) ) ;
#121943=CONICAL_SURFACE ( 'NONE', #48891, 0.09999999999999982514, 0.003490658503988666988 ) ;
#121944=CARTESIAN_POINT ( 'NONE',  ( 8.349999999999919709, 12.50000000000000000, 6.495190528383297135 ) ) ;
#121945=DIRECTION ( 'NONE',  ( 0.000000000000000000, -0.9999939076577903929, 0.003490651415223739937 ) ) ;
#121946=AXIS2_PLACEMENT_3D ( 'NONE', #100024, #90170, #40473 ) ;
#121947=CARTESIAN_POINT ( 'NONE',  ( 6.449999999999930012, 12.50000000000000000, -1.883746621131363597 ) ) ;
#121948=DIRECTION ( 'NONE',  ( -0.000000000000000000, -1.000000000000000000, -0.000000000000000000 ) ) ;
#121949=CIRCLE ( 'NONE', #75965, 0.06509327318403745899 ) ;
#121950=CONICAL_SURFACE ( 'NONE', #67649, 0.09999999999999982514, 0.003490658503988666988 ) ;
#121951=ORIENTED_EDGE ( 'NONE', *, *, #121641, .F. ) ;
#121952=CARTESIAN_POINT ( 'NONE',  ( -13.14999999999999147, 2.500000000000000000, -2.511473670974875727 ) ) ;
#121953=ADVANCED_FACE ( 'NONE', ( #16793 ), #100621, .T. ) ;
#121954=ORIENTED_EDGE ( 'NONE', *, *, #85160, .T. ) ;
#121955=CARTESIAN_POINT ( 'NONE',  ( 7.299999999999927880, 2.500000000000000000, 3.883716857408421319 ) ) ;
#121956=CONICAL_SURFACE ( 'NONE', #111480, 0.1000000000000002554, 0.003490658503988666988 ) ;
#121957=ORIENTED_EDGE ( 'NONE', *, *, #125056, .T. ) ;
#121958=AXIS2_PLACEMENT_3D ( 'NONE', #73473, #95067, #53850 ) ;
#121959=PLANE ( 'NONE',  #44738 ) ;
#121960=ORIENTED_EDGE ( 'NONE', *, *, #115363, .T. ) ;
#121961=ADVANCED_FACE ( 'NONE', ( #75106 ), #25339, .T. ) ;
#121962=CARTESIAN_POINT ( 'NONE',  ( 12.49999999999993605, 2.500000000000000000, -2.276824562219559311E-15 ) ) ;
#121963=DIRECTION ( 'NONE',  ( 0.000000000000000000, -0.9999939076577903929, 0.003490651415223739937 ) ) ;
#121964=ORIENTED_EDGE ( 'NONE', *, *, #50975, .T. ) ;
#121965=EDGE_CURVE ( 'NONE', #2395, #12221, #94370, .T. ) ;
#121966=ADVANCED_FACE ( 'NONE', ( #9586 ), #50020, .T. ) ;
#121967=ORIENTED_EDGE ( 'NONE', *, *, #82673, .T. ) ;
#121968=DIRECTION ( 'NONE',  ( 0.000000000000000000, 0.000000000000000000, 1.000000000000000000 ) ) ;
#121969=DIRECTION ( 'NONE',  ( -0.000000000000000000, -1.000000000000000000, -0.000000000000000000 ) ) ;
#121970=EDGE_CURVE ( 'NONE', #40079, #98189, #117570, .T. ) ;
#121971=DIRECTION ( 'NONE',  ( -0.000000000000000000, 1.000000000000000000, -0.000000000000000000 ) ) ;
#121972=EDGE_CURVE ( 'NONE', #124183, #1645, #45520, .T. ) ;
#121973=DIRECTION ( 'NONE',  ( -0.000000000000000000, -1.000000000000000000, -0.000000000000000000 ) ) ;
#121974=VECTOR ( 'NONE', #108151, 1000.000000000000000 ) ;
#121975=CARTESIAN_POINT ( 'NONE',  ( -8.100000000000013856, 12.50000000000000000, -3.918623584224389056 ) ) ;
#121976=ORIENTED_EDGE ( 'NONE', *, *, #14099, .F. ) ;
#121977=CARTESIAN_POINT ( 'NONE',  ( 2.500000000000001332, -2.392226903609812272, 9.521986658763283984 ) ) ;
#121978=ADVANCED_FACE ( 'NONE', ( #67852 ), #114738, .T. ) ;
#121979=CIRCLE ( 'NONE', #109450, 0.06509327318403745899 ) ;
#121980=VERTEX_POINT ( 'NONE', #99267 ) ;
#121981=EDGE_CURVE ( 'NONE', #71812, #35395, #98584, .T. ) ;
#121982=FACE_OUTER_BOUND ( 'NONE', #77629, .T. ) ;
#121983=PLANE ( 'NONE',  #91838 ) ;
#121984=CONICAL_SURFACE ( 'NONE', #69744, 0.09999999999999982514, 0.003490658503988666988 ) ;
#121985=EDGE_CURVE ( 'NONE', #56742, #27176, #80266, .T. ) ;
#121986=CARTESIAN_POINT ( 'NONE',  ( 3.099999999999945022, 12.50000000000000000, -0.3464101615137783474 ) ) ;
#121987=FACE_OUTER_BOUND ( 'NONE', #116634, .T. ) ;
#121988=FACE_OUTER_BOUND ( 'NONE', #72500, .T. ) ;
#121990=DIRECTION ( 'NONE',  ( -4.274815082592931898E-19, -0.9999939076577903929, -0.003490651415223739937 ) ) ;
#121991=VECTOR ( 'NONE', #48876, 1000.000000000000000 ) ;
#121993=AXIS2_PLACEMENT_3D ( 'NONE', #6930, #86807, #48837 ) ;
#121994=AXIS2_PLACEMENT_3D ( 'NONE', #38451, #78373, #118273 ) ;
#121995=CARTESIAN_POINT ( 'NONE',  ( 4.599999999999940137, 2.500000000000000000, -4.922947341949753586 ) ) ;
#121996=DIRECTION ( 'NONE',  ( 0.000000000000000000, 0.000000000000000000, 1.000000000000000000 ) ) ;
#121997=DIRECTION ( 'NONE',  ( -0.000000000000000000, 1.000000000000000000, -0.000000000000000000 ) ) ;
#121998=EDGE_LOOP ( 'NONE', ( #88600, #54566, #13279, #39825 ) ) ;
#121999=AXIS2_PLACEMENT_3D ( 'NONE', #15470, #75676, #16744 ) ;
#122000=EDGE_LOOP ( 'NONE', ( #113528, #127447 ) ) ;
#122001=DIRECTION ( 'NONE',  ( 0.000000000000000000, 1.000000000000000000, 0.000000000000000000 ) ) ;
#122002=VERTEX_POINT ( 'NONE', #57399 ) ;
#122003=CIRCLE ( 'NONE', #21657, 0.06509327318403745899 ) ;
#122004=CIRCLE ( 'NONE', #94904, 0.06509327318403745899 ) ;
#122005=ORIENTED_EDGE ( 'NONE', *, *, #74986, .T. ) ;
#122006=CIRCLE ( 'NONE', #119945, 0.1000000000000000056 ) ;
#122007=DIRECTION ( 'NONE',  ( -0.000000000000000000, 1.000000000000000000, -0.000000000000000000 ) ) ;
#122008=VECTOR ( 'NONE', #33667, 1000.000000000000000 ) ;
#122009=VERTEX_POINT ( 'NONE', #97957 ) ;
#122010=DIRECTION ( 'NONE',  ( 0.000000000000000000, 0.000000000000000000, 1.000000000000000000 ) ) ;
#122011=FACE_OUTER_BOUND ( 'NONE', #6423, .T. ) ;
#122012=CARTESIAN_POINT ( 'NONE',  ( 17.84432265422787722, 2.533187527836262554, 5.021315468706709417 ) ) ;
#122013=CIRCLE ( 'NONE', #109485, 0.1000000000000000056 ) ;
#122014=EDGE_LOOP ( 'NONE', ( #44381, #105444 ) ) ;
#122015=DIRECTION ( 'NONE',  ( -4.274815082592931898E-19, -0.9999939076577903929, -0.003490651415223739937 ) ) ;
#122016=CARTESIAN_POINT ( 'NONE',  ( 12.29999999999990301, 2.500000000000000000, -0.2464101615137782308 ) ) ;
#122017=ADVANCED_FACE ( 'NONE', ( #97321 ), #7635, .T. ) ;
#122018=ORIENTED_EDGE ( 'NONE', *, *, #117414, .T. ) ;
#122019=EDGE_CURVE ( 'NONE', #77678, #39357, #12332, .T. ) ;
#122020=ORIENTED_EDGE ( 'NONE', *, *, #45192, .T. ) ;
#122021=ADVANCED_FACE ( 'NONE', ( #68495 ), #112694, .T. ) ;
#122022=VERTEX_POINT ( 'NONE', #20062 ) ;
#122023=DIRECTION ( 'NONE',  ( 0.000000000000000000, 1.000000000000000000, 0.000000000000000000 ) ) ;
#122024=DIRECTION ( 'NONE',  ( 0.000000000000000000, 1.000000000000000000, 0.000000000000000000 ) ) ;
#122025=CONICAL_SURFACE ( 'NONE', #40571, 0.1000000000000002554, 0.003490658503988666988 ) ;
#122026=CARTESIAN_POINT ( 'NONE',  ( -10.00000000000000711, 2.500000000000000000, -3.637306695894645614 ) ) ;
#122027=CIRCLE ( 'NONE', #109504, 0.1000000000000000472 ) ;
#122028=FACE_BOUND ( 'NONE', #39648, .T. ) ;
#122029=ORIENTED_EDGE ( 'NONE', *, *, #65033, .F. ) ;
#122030=DIRECTION ( 'NONE',  ( 0.000000000000000000, 1.000000000000000000, 0.000000000000000000 ) ) ;
#122031=CARTESIAN_POINT ( 'NONE',  ( -1.050000000000038680, 12.50000000000000000, 6.841600689897072485 ) ) ;
#122032=ORIENTED_EDGE ( 'NONE', *, *, #49969, .F. ) ;
#122033=EDGE_CURVE ( 'NONE', #36138, #11513, #93823, .T. ) ;
#122034=CARTESIAN_POINT ( 'NONE',  ( -2.500000000000032863, 2.500000000000000000, 5.022947341949748790 ) ) ;
#122035=AXIS2_PLACEMENT_3D ( 'NONE', #129271, #39603, #79507 ) ;
#122036=CARTESIAN_POINT ( 'NONE',  ( -7.100000000000013856, 12.50000000000000000, 5.022947341949748790 ) ) ;
#122037=VECTOR ( 'NONE', #99995, 1000.000000000000000 ) ;
#122038=CIRCLE ( 'NONE', #67642, 0.06509327318403745899 ) ;
#122039=PLANE ( 'NONE',  #67426 ) ;
#122040=CONICAL_SURFACE ( 'NONE', #103257, 0.09999999999999982514, 0.003490658503988666988 ) ;
#122041=CARTESIAN_POINT ( 'NONE',  ( -0.6500000000000403233, 2.500000000000000000, 6.148780366869520009 ) ) ;
#122042=CARTESIAN_POINT ( 'NONE',  ( 11.69999999999990870, 2.500000000000000000, 4.330127018922196314 ) ) ;
#122043=FACE_OUTER_BOUND ( 'NONE', #32221, .T. ) ;
#122044=DIRECTION ( 'NONE',  ( 0.000000000000000000, -0.9999939076577903929, 0.003490651415223739937 ) ) ;
#122045=AXIS2_PLACEMENT_3D ( 'NONE', #116596, #47236, #66207 ) ;
#122046=VECTOR ( 'NONE', #2232, 1000.000000000000000 ) ;
#122047=ORIENTED_EDGE ( 'NONE', *, *, #61431, .F. ) ;
#122048=EDGE_LOOP ( 'NONE', ( #124295, #2186, #69441, #15371 ) ) ;
#122049=ORIENTED_EDGE ( 'NONE', *, *, #26019, .F. ) ;
#122050=ORIENTED_EDGE ( 'NONE', *, *, #72324, .T. ) ;
#122051=DIRECTION ( 'NONE',  ( 0.000000000000000000, 0.000000000000000000, 1.000000000000000000 ) ) ;
#122052=CARTESIAN_POINT ( 'NONE',  ( -1.250000000000035749, 12.50000000000000000, -7.122917578226816815 ) ) ;
#122053=AXIS2_PLACEMENT_3D ( 'NONE', #83166, #63522, #3938 ) ;
#122054=DIRECTION ( 'NONE',  ( 0.000000000000000000, 1.000000000000000000, 0.000000000000000000 ) ) ;
#122055=ORIENTED_EDGE ( 'NONE', *, *, #2588, .F. ) ;
#122056=FACE_BOUND ( 'NONE', #111071, .T. ) ;
#122057=EDGE_CURVE ( 'NONE', #46303, #48905, #39721, .T. ) ;
#122058=CARTESIAN_POINT ( 'NONE',  ( -13.14999999999999147, 12.50000000000000000, 2.511473670974877503 ) ) ;
#122059=DIRECTION ( 'NONE',  ( 0.000000000000000000, -0.000000000000000000, 1.000000000000000000 ) ) ;
#122060=LINE ( 'NONE', #61853, #15685 ) ;
#122061=CARTESIAN_POINT ( 'NONE',  ( -9.200000000000009948, 2.500000000000000000, -4.330127018922197202 ) ) ;
#122062=CARTESIAN_POINT ( 'NONE',  ( 11.64999999999990443, 12.50000000000000000, 1.472243186433545459 ) ) ;
#122063=DIRECTION ( 'NONE',  ( 0.000000000000000000, 0.000000000000000000, 1.000000000000000000 ) ) ;
#122065=DIRECTION ( 'NONE',  ( 0.000000000000000000, 1.000000000000000000, 0.000000000000000000 ) ) ;
#122066=DIRECTION ( 'NONE',  ( -0.000000000000000000, 1.000000000000000000, -0.000000000000000000 ) ) ;
#122068=AXIS2_PLACEMENT_3D ( 'NONE', #54386, #91741, #81909 ) ;
#122069=ORIENTED_EDGE ( 'NONE', *, *, #22038, .F. ) ;
#122070=ORIENTED_EDGE ( 'NONE', *, *, #127538, .F. ) ;
#122071=EDGE_LOOP ( 'NONE', ( #55052, #98645 ) ) ;
#122072=EDGE_CURVE ( 'NONE', #59946, #37252, #104287, .T. ) ;
#122073=ORIENTED_EDGE ( 'NONE', *, *, #94102, .F. ) ;
#122074=ORIENTED_EDGE ( 'NONE', *, *, #45305, .F. ) ;
#122075=EDGE_LOOP ( 'NONE', ( #15150, #41778 ) ) ;
#122076=DIRECTION ( 'NONE',  ( 0.000000000000000000, 0.000000000000000000, -1.000000000000000000 ) ) ;
#122077=ORIENTED_EDGE ( 'NONE', *, *, #2706, .F. ) ;
#122078=ORIENTED_EDGE ( 'NONE', *, *, #21353, .F. ) ;
#122079=VECTOR ( 'NONE', #29324, 1000.000000000000000 ) ;
#122080=AXIS2_PLACEMENT_3D ( 'NONE', #65495, #5913, #26234 ) ;
#122081=DIRECTION ( 'NONE',  ( 0.000000000000000000, 0.000000000000000000, -1.000000000000000000 ) ) ;
#122082=DIRECTION ( 'NONE',  ( 0.000000000000000000, 1.000000000000000000, 0.000000000000000000 ) ) ;
#122083=DIRECTION ( 'NONE',  ( 0.000000000000000000, -0.000000000000000000, 1.000000000000000000 ) ) ;
#122084=FACE_OUTER_BOUND ( 'NONE', #46881, .T. ) ;
#122085=EDGE_CURVE ( 'NONE', #79702, #112590, #72982, .T. ) ;
#122086=AXIS2_PLACEMENT_3D ( 'NONE', #54874, #16857, #75802 ) ;
#122087=VERTEX_POINT ( 'NONE', #90061 ) ;
#122088=DIRECTION ( 'NONE',  ( -0.000000000000000000, -1.000000000000000000, -0.000000000000000000 ) ) ;
#122089=CIRCLE ( 'NONE', #105356, 0.1000000000000002554 ) ;
#122090=EDGE_LOOP ( 'NONE', ( #110076, #78040 ) ) ;
#122091=AXIS2_PLACEMENT_3D ( 'NONE', #112332, #100563, #50832 ) ;
#122092=ORIENTED_EDGE ( 'NONE', *, *, #4062, .F. ) ;
#122093=CARTESIAN_POINT ( 'NONE',  ( 0.8499999999999527933, 2.500000000000000000, 7.288010851410849256 ) ) ;
#122094=DIRECTION ( 'NONE',  ( 0.000000000000000000, 1.000000000000000000, 0.000000000000000000 ) ) ;
#122095=ADVANCED_FACE ( 'NONE', ( #39072 ), #87481, .T. ) ;
#122096=ORIENTED_EDGE ( 'NONE', *, *, #39824, .F. ) ;
#122097=VERTEX_POINT ( 'NONE', #118245 ) ;
#122098=DIRECTION ( 'NONE',  ( 0.000000000000000000, 1.000000000000000000, 0.000000000000000000 ) ) ;
#122099=PLANE ( 'NONE',  #49579 ) ;
#122100=AXIS2_PLACEMENT_3D ( 'NONE', #109454, #108792, #19792 ) ;
#122101=DIRECTION ( 'NONE',  ( 0.000000000000000000, 0.000000000000000000, -1.000000000000000000 ) ) ;
#122102=CIRCLE ( 'NONE', #48945, 0.1000000000000002554 ) ;
#122103=AXIS2_PLACEMENT_3D ( 'NONE', #97696, #59078, #47975 ) ;
#122104=CARTESIAN_POINT ( 'NONE',  ( -9.600000000000008527, 12.50000000000000000, -3.637306695894645614 ) ) ;
#122105=LINE ( 'NONE', #120805, #56533 ) ;
#122106=CIRCLE ( 'NONE', #119949, 0.1000000000000002554 ) ;
#122107=EDGE_LOOP ( 'NONE', ( #91168, #51589 ) ) ;
#122108=AXIS2_PLACEMENT_3D ( 'NONE', #31238, #22708, #71798 ) ;
#122109=CARTESIAN_POINT ( 'NONE',  ( 1.049999999999952971, 2.500000000000000000, 6.048780366869521252 ) ) ;
#122110=EDGE_LOOP ( 'NONE', ( #78556, #62364, #90132, #124514 ) ) ;
#122111=CARTESIAN_POINT ( 'NONE',  ( 87.50000000000002842, 7.032605354647524010, 2.693424153406289712 ) ) ;
#122112=EDGE_CURVE ( 'NONE', #120532, #62968, #127431, .T. ) ;
#122113=CARTESIAN_POINT ( 'NONE',  ( 4.799999999999934097, 2.500000000000000000, 4.776537180435972196 ) ) ;
#122114=CARTESIAN_POINT ( 'NONE',  ( 8.749999999999921840, 2.500000000000000000, 2.757883832488649656 ) ) ;
#122115=CARTESIAN_POINT ( 'NONE',  ( 15.19999999999989271, 2.500000000000000000, -0.2464101615137783419 ) ) ;
#122116=DIRECTION ( 'NONE',  ( 0.000000000000000000, 0.000000000000000000, -1.000000000000000000 ) ) ;
#122117=EDGE_LOOP ( 'NONE', ( #79335, #2065, #85997, #121530 ) ) ;
#122118=EDGE_CURVE ( 'NONE', #64939, #9837, #19386, .T. ) ;
#122119=DIRECTION ( 'NONE',  ( 0.000000000000000000, -0.9999939076577903929, 0.003490651415223739937 ) ) ;
#122120=VECTOR ( 'NONE', #127438, 1000.000000000000000 ) ;
#122121=DIRECTION ( 'NONE',  ( 0.000000000000000000, -0.000000000000000000, 1.000000000000000000 ) ) ;
#122122=ORIENTED_EDGE ( 'NONE', *, *, #4002, .F. ) ;
#122123=ORIENTED_EDGE ( 'NONE', *, *, #65311, .F. ) ;
#122124=AXIS2_PLACEMENT_3D ( 'NONE', #61912, #103105, #33722 ) ;
#122125=ADVANCED_FACE ( 'NONE', ( #92656 ), #14458, .T. ) ;
#122126=CIRCLE ( 'NONE', #117898, 0.06509327318403741736 ) ;
#122127=EDGE_CURVE ( 'NONE', #24551, #12644, #6062, .T. ) ;
#122128=ORIENTED_EDGE ( 'NONE', *, *, #89257, .T. ) ;
#122129=CARTESIAN_POINT ( 'NONE',  ( 17.50000000000000000, 0.9166666666666684060, 3.432456362931491700 ) ) ;
#122130=CARTESIAN_POINT ( 'NONE',  ( 1.249999999999952038, 2.500000000000000000, -1.472243186433550122 ) ) ;
#122131=ADVANCED_FACE ( 'NONE', ( #32480 ), #83497, .T. ) ;
#122133=EDGE_CURVE ( 'NONE', #63089, #25747, #29088, .T. ) ;
#122134=CARTESIAN_POINT ( 'NONE',  ( -0.4000000000000396572, 2.500000000000000000, 4.430127018922196847 ) ) ;
#122135=DIRECTION ( 'NONE',  ( 0.000000000000000000, 0.000000000000000000, -1.000000000000000000 ) ) ;
#122136=AXIS2_PLACEMENT_3D ( 'NONE', #87215, #105588, #35562 ) ;
#122137=AXIS2_PLACEMENT_3D ( 'NONE', #12790, #73022, #104414 ) ;
#122138=CARTESIAN_POINT ( 'NONE',  ( 5.849999999999933031, 2.500000000000000000, -1.372243186433550033 ) ) ;
#122139=VECTOR ( 'NONE', #31050, 1000.000000000000000 ) ;
#122140=CARTESIAN_POINT ( 'NONE',  ( 7.949999999999925571, 12.50000000000000000, -6.495190528383302464 ) ) ;
#122141=VECTOR ( 'NONE', #30505, 1000.000000000000000 ) ;
#122142=ADVANCED_FACE ( 'NONE', ( #93305 ), #24863, .T. ) ;
#122143=ADVANCED_FACE ( 'NONE', ( #122763 ), #63198, .T. ) ;
#122144=EDGE_CURVE ( 'NONE', #11888, #46085, #75037, .T. ) ;
#122145=EDGE_CURVE ( 'NONE', #181, #104766, #13438, .T. ) ;
#122146=CIRCLE ( 'NONE', #69999, 0.1000000000000002554 ) ;
#122147=CARTESIAN_POINT ( 'NONE',  ( 2.899999999999946620, 12.50000000000000000, 0.6928203230275494784 ) ) ;
#122148=CIRCLE ( 'NONE', #3008, 0.06509327318403745899 ) ;
#122149=EDGE_CURVE ( 'NONE', #62966, #70666, #73017, .T. ) ;
#122150=ORIENTED_EDGE ( 'NONE', *, *, #32448, .F. ) ;
#122151=DIRECTION ( 'NONE',  ( 0.000000000000000000, 0.000000000000000000, 1.000000000000000000 ) ) ;
#122152=AXIS2_PLACEMENT_3D ( 'NONE', #80432, #79149, #100688 ) ;
#122153=DIRECTION ( 'NONE',  ( -0.000000000000000000, 1.000000000000000000, -0.000000000000000000 ) ) ;
#122154=DIRECTION ( 'NONE',  ( 0.000000000000000000, 0.000000000000000000, 1.000000000000000000 ) ) ;
#122155=DIRECTION ( 'NONE',  ( 0.000000000000000000, 1.000000000000000000, 0.000000000000000000 ) ) ;
#122156=ADVANCED_FACE ( 'NONE', ( #110357 ), #43659, .T. ) ;
#122157=ORIENTED_EDGE ( 'NONE', *, *, #47155, .T. ) ;
#122158=LINE ( 'NONE', #32497, #46737 ) ;
#122159=FACE_OUTER_BOUND ( 'NONE', #121017, .T. ) ;
#122160=CARTESIAN_POINT ( 'NONE',  ( 0.7999999999999553024, 2.500000000000000000, -4.330127018922201643 ) ) ;
#122161=ORIENTED_EDGE ( 'NONE', *, *, #24505, .T. ) ;
#122162=AXIS2_PLACEMENT_3D ( 'NONE', #127434, #27281, #67179 ) ;
#122163=ORIENTED_EDGE ( 'NONE', *, *, #34732, .T. ) ;
#122164=LINE ( 'NONE', #90751, #7036 ) ;
#122165=ORIENTED_EDGE ( 'NONE', *, *, #46463, .F. ) ;
#122166=VERTEX_POINT ( 'NONE', #20700 ) ;
#122167=DIRECTION ( 'NONE',  ( 0.000000000000000000, 1.000000000000000000, 0.000000000000000000 ) ) ;
#122168=CARTESIAN_POINT ( 'NONE',  ( -10.00000000000000533, 2.500000000000000000, -5.022947341949749678 ) ) ;
#122169=CARTESIAN_POINT ( 'NONE',  ( 7.699999999999923794, 2.500000000000000000, -3.883716857408426648 ) ) ;
#122170=CARTESIAN_POINT ( 'NONE',  ( -14.59999999999998366, 12.50000000000000000, -0.6928203230275520319 ) ) ;
#122171=AXIS2_PLACEMENT_3D ( 'NONE', #42514, #62150, #3222 ) ;
#122172=ORIENTED_EDGE ( 'NONE', *, *, #87055, .F. ) ;
#122173=CARTESIAN_POINT ( 'NONE',  ( -2.300000000000032685, 12.50000000000000000, -4.676537180435978769 ) ) ;
#122174=ORIENTED_EDGE ( 'NONE', *, *, #36442, .T. ) ;
#122175=DIRECTION ( 'NONE',  ( 0.000000000000000000, 0.000000000000000000, 1.000000000000000000 ) ) ;
#122176=CARTESIAN_POINT ( 'NONE',  ( -5.400000000000019895, 12.50000000000000000, 4.395220292106234439 ) ) ;
#122177=VERTEX_POINT ( 'NONE', #50804 ) ;
#122178=EDGE_CURVE ( 'NONE', #18500, #107528, #60637, .T. ) ;
#122179=ORIENTED_EDGE ( 'NONE', *, *, #86344, .T. ) ;
#122180=EDGE_CURVE ( 'NONE', #70884, #108643, #116788, .T. ) ;
#122181=EDGE_LOOP ( 'NONE', ( #3020, #121976, #116699, #103195 ) ) ;
#122182=VERTEX_POINT ( 'NONE', #94576 ) ;
#122183=DIRECTION ( 'NONE',  ( 0.000000000000000000, 0.000000000000000000, 1.000000000000000000 ) ) ;
#122184=CARTESIAN_POINT ( 'NONE',  ( 14.66596006039175748, 2.500000000000513811, 7.515560524214964566 ) ) ;
#122185=CARTESIAN_POINT ( 'NONE',  ( -6.900000000000015454, 2.500000000000000000, 4.776537180435972196 ) ) ;
#122186=FACE_BOUND ( 'NONE', #15668, .T. ) ;
#122187=ORIENTED_EDGE ( 'NONE', *, *, #125677, .T. ) ;
#122189=DIRECTION ( 'NONE',  ( -0.000000000000000000, 1.000000000000000000, -0.000000000000000000 ) ) ;
#122190=CARTESIAN_POINT ( 'NONE',  ( 4.599999999999938360, 12.50000000000000000, 0.06509327318403515528 ) ) ;
#122191=ADVANCED_FACE ( 'NONE', ( #95242 ), #86032, .T. ) ;
#122192=VECTOR ( 'NONE', #54391, 1000.000000000000000 ) ;
#122193=AXIS2_PLACEMENT_3D ( 'NONE', #116239, #26586, #75038 ) ;
#122194=FACE_OUTER_BOUND ( 'NONE', #44510, .T. ) ;
#122195=DIRECTION ( 'NONE',  ( 0.000000000000000000, 0.000000000000000000, -1.000000000000000000 ) ) ;
#122196=AXIS2_PLACEMENT_3D ( 'NONE', #22420, #101613, #119957 ) ;
#122197=CARTESIAN_POINT ( 'NONE',  ( 13.34999999999989662, 12.50000000000000000, -1.407149913249512663 ) ) ;
#122198=AXIS2_PLACEMENT_3D ( 'NONE', #116210, #6881, #63906 ) ;
#122199=CARTESIAN_POINT ( 'NONE',  ( 9.149999999999918643, 2.500000000000000000, -6.495190528383302464 ) ) ;
#122200=ORIENTED_EDGE ( 'NONE', *, *, #49089, .F. ) ;
#122201=VERTEX_POINT ( 'NONE', #36339 ) ;
#122202=ORIENTED_EDGE ( 'NONE', *, *, #21939, .F. ) ;
#122203=ORIENTED_EDGE ( 'NONE', *, *, #118860, .T. ) ;
#122204=ORIENTED_EDGE ( 'NONE', *, *, #56333, .F. ) ;
#122205=FACE_OUTER_BOUND ( 'NONE', #97110, .T. ) ;
#122206=CARTESIAN_POINT ( 'NONE',  ( -7.100000000000013856, 12.50000000000000000, 5.022947341949748790 ) ) ;
#122207=EDGE_LOOP ( 'NONE', ( #119693, #5643 ) ) ;
#122208=FACE_BOUND ( 'NONE', #11766, .T. ) ;
#122209=FACE_OUTER_BOUND ( 'NONE', #8895, .T. ) ;
#122210=AXIS2_PLACEMENT_3D ( 'NONE', #10386, #98754, #91531 ) ;
#122211=CIRCLE ( 'NONE', #78310, 0.06509327318403745899 ) ;
#122212=AXIS2_PLACEMENT_3D ( 'NONE', #125958, #105025, #26490 ) ;
#122213=EDGE_LOOP ( 'NONE', ( #112721, #95319, #13830, #115229 ) ) ;
#122214=AXIS2_PLACEMENT_3D ( 'NONE', #42738, #4056, #11948 ) ;
#122215=CARTESIAN_POINT ( 'NONE',  ( 4.599999999999938360, 12.50000000000000000, -0.6928203230275541413 ) ) ;
#122216=CARTESIAN_POINT ( 'NONE',  ( -13.34999999999999076, 2.500000000000000000, -2.165063509461099489 ) ) ;
#122217=DIRECTION ( 'NONE',  ( 0.000000000000000000, 0.000000000000000000, 1.000000000000000000 ) ) ;
#122218=EDGE_LOOP ( 'NONE', ( #63079, #38759 ) ) ;
#122219=DIRECTION ( 'NONE',  ( 0.000000000000000000, 0.000000000000000000, 1.000000000000000000 ) ) ;
#122220=EDGE_CURVE ( 'NONE', #102068, #25999, #121006, .T. ) ;
#122221=AXIS2_PLACEMENT_3D ( 'NONE', #3770, #1826, #124191 ) ;
#122222=VERTEX_POINT ( 'NONE', #64478 ) ;
#122224=AXIS2_PLACEMENT_3D ( 'NONE', #114095, #63711, #64976 ) ;
#122225=ORIENTED_EDGE ( 'NONE', *, *, #128228, .F. ) ;
#122226=ORIENTED_EDGE ( 'NONE', *, *, #230, .T. ) ;
#122227=DIRECTION ( 'NONE',  ( 0.000000000000000000, 0.000000000000000000, 1.000000000000000000 ) ) ;
#122228=CIRCLE ( 'NONE', #72060, 0.06509327318403745899 ) ;
#122229=DIRECTION ( 'NONE',  ( 0.000000000000000000, -0.000000000000000000, 1.000000000000000000 ) ) ;
#122230=FACE_OUTER_BOUND ( 'NONE', #54118, .T. ) ;
#122231=ORIENTED_EDGE ( 'NONE', *, *, #23284, .T. ) ;
#122232=DIRECTION ( 'NONE',  ( 0.000000000000000000, 1.000000000000000000, 0.000000000000000000 ) ) ;
#122233=AXIS2_PLACEMENT_3D ( 'NONE', #23413, #104561, #5062 ) ;
#122234=AXIS2_PLACEMENT_3D ( 'NONE', #54269, #24163, #14947 ) ;
#122235=DIRECTION ( 'NONE',  ( -0.000000000000000000, 1.000000000000000000, -0.000000000000000000 ) ) ;
#122236=DIRECTION ( 'NONE',  ( -0.000000000000000000, -1.000000000000000000, -0.000000000000000000 ) ) ;
#122237=DIRECTION ( 'NONE',  ( 0.000000000000000000, 0.000000000000000000, -1.000000000000000000 ) ) ;
#122240=ORIENTED_EDGE ( 'NONE', *, *, #11897, .T. ) ;
#122241=EDGE_CURVE ( 'NONE', #83886, #94318, #4901, .T. ) ;
#122242=FACE_OUTER_BOUND ( 'NONE', #121310, .T. ) ;
#122244=ORIENTED_EDGE ( 'NONE', *, *, #6011, .T. ) ;
#122245=DIRECTION ( 'NONE',  ( 0.000000000000000000, -0.000000000000000000, 1.000000000000000000 ) ) ;
#122246=VERTEX_POINT ( 'NONE', #74954 ) ;
#122247=ORIENTED_EDGE ( 'NONE', *, *, #120225, .F. ) ;
#122248=DIRECTION ( 'NONE',  ( 0.000000000000000000, 0.000000000000000000, 1.000000000000000000 ) ) ;
#122249=CARTESIAN_POINT ( 'NONE',  ( 12.09999999999990550, 2.500000000000000000, 3.637306695894644726 ) ) ;
#122250=CARTESIAN_POINT ( 'NONE',  ( -9.999999999999971578, 12.50000000000000000, -4.265033745738159965 ) ) ;
#122251=CARTESIAN_POINT ( 'NONE',  ( -13.34999999999999076, 2.500000000000000000, -1.472243186433547901 ) ) ;
#122252=EDGE_CURVE ( 'NONE', #79726, #35730, #91754, .T. ) ;
#122253=CARTESIAN_POINT ( 'NONE',  ( 3.349999999999945466, 12.50000000000000000, -6.430097255199264339 ) ) ;
#122254=CONICAL_SURFACE ( 'NONE', #11423, 0.09999999999999982514, 0.003490658503988666988 ) ;
#122255=EDGE_LOOP ( 'NONE', ( #40778, #15171, #51508, #72284 ) ) ;
#122256=ORIENTED_EDGE ( 'NONE', *, *, #61565, .F. ) ;
#122257=DIRECTION ( 'NONE',  ( 0.000000000000000000, -0.000000000000000000, 1.000000000000000000 ) ) ;
#122258=FACE_OUTER_BOUND ( 'NONE', #8388, .T. ) ;
#122259=DIRECTION ( 'NONE',  ( -0.000000000000000000, -1.000000000000000000, -0.000000000000000000 ) ) ;
#122260=ORIENTED_EDGE ( 'NONE', *, *, #11237, .F. ) ;
#122261=VERTEX_POINT ( 'NONE', #105707 ) ;
#122262=DIRECTION ( 'NONE',  ( 0.000000000000000000, -0.000000000000000000, 1.000000000000000000 ) ) ;
#122263=CIRCLE ( 'NONE', #49021, 0.06509327318403745899 ) ;
#122264=VERTEX_POINT ( 'NONE', #103773 ) ;
#122265=DIRECTION ( 'NONE',  ( 0.000000000000000000, 1.000000000000000000, 0.000000000000000000 ) ) ;
#122266=CARTESIAN_POINT ( 'NONE',  ( -0.6000000000000383915, 2.500000000000000000, -3.983716857408426293 ) ) ;
#122267=CIRCLE ( 'NONE', #107677, 0.09999999999999982514 ) ;
#122268=LINE ( 'NONE', #11653, #109607 ) ;
#122269=ORIENTED_EDGE ( 'NONE', *, *, #69248, .F. ) ;
#122270=DIRECTION ( 'NONE',  ( -0.000000000000000000, -1.000000000000000000, -0.000000000000000000 ) ) ;
#122271=DIRECTION ( 'NONE',  ( -4.274815082592931898E-19, -0.9999939076577903929, -0.003490651415223739937 ) ) ;
#122272=CARTESIAN_POINT ( 'NONE',  ( -7.500000000000001776, 1.500000000000000000, 1.734723475976807094E-15 ) ) ;
#122273=CARTESIAN_POINT ( 'NONE',  ( -15.19999999999998330, 12.50000000000000000, 0.3464101615137758494 ) ) ;
#122274=PLANE ( 'NONE',  #72952 ) ;
#122275=EDGE_LOOP ( 'NONE', ( #32400, #126879, #88664, #32811 ) ) ;
#122276=AXIS2_PLACEMENT_3D ( 'NONE', #102987, #5430, #54524 ) ;
#122278=CARTESIAN_POINT ( 'NONE',  ( 9.149999999999916866, 12.50000000000000000, 7.188010851410848723 ) ) ;
#122279=DIRECTION ( 'NONE',  ( 0.000000000000000000, 0.000000000000000000, -1.000000000000000000 ) ) ;
#122280=AXIS2_PLACEMENT_3D ( 'NONE', #35288, #66016, #116394 ) ;
#122281=VERTEX_POINT ( 'NONE', #104410 ) ;
#122282=ORIENTED_EDGE ( 'NONE', *, *, #43960, .F. ) ;
#122283=EDGE_CURVE ( 'NONE', #124086, #22468, #108473, .T. ) ;
#122285=DIRECTION ( 'NONE',  ( -0.000000000000000000, -1.000000000000000000, -0.000000000000000000 ) ) ;
#122286=DIRECTION ( 'NONE',  ( -0.000000000000000000, 1.000000000000000000, -0.000000000000000000 ) ) ;
#122287=EDGE_CURVE ( 'NONE', #125928, #95328, #33292, .T. ) ;
#122288=CARTESIAN_POINT ( 'NONE',  ( -10.85000000000000142, 2.500000000000000000, -2.857883832488649745 ) ) ;
#122289=CARTESIAN_POINT ( 'NONE',  ( 4.399999999999939071, 2.500000000000000000, 0.4464101615137736623 ) ) ;
#122290=AXIS2_PLACEMENT_3D ( 'NONE', #97539, #127019, #37351 ) ;
#122291=CARTESIAN_POINT ( 'NONE',  ( 5.849999999999933920, 12.50000000000000000, 5.802370205355744659 ) ) ;
#122292=CIRCLE ( 'NONE', #86758, 0.09999999999999982514 ) ;
#122293=CARTESIAN_POINT ( 'NONE',  ( 2.699999999999946443, 12.50000000000000000, -4.048810130592463530 ) ) ;
#122294=LINE ( 'NONE', #11016, #49830 ) ;
#122295=EDGE_CURVE ( 'NONE', #58087, #96104, #125969, .T. ) ;
#122296=ADVANCED_FACE ( 'NONE', ( #66409 ), #20667, .T. ) ;
#122297=ADVANCED_FACE ( 'NONE', ( #14073 ), #112414, .T. ) ;
#122298=FACE_OUTER_BOUND ( 'NONE', #68330, .T. ) ;
#122299=ORIENTED_EDGE ( 'NONE', *, *, #90083, .T. ) ;
#122300=VERTEX_POINT ( 'NONE', #75580 ) ;
#122301=ADVANCED_FACE ( 'NONE', ( #126636 ), #47666, .T. ) ;
#122302=ORIENTED_EDGE ( 'NONE', *, *, #79472, .F. ) ;
#122303=ORIENTED_EDGE ( 'NONE', *, *, #51701, .T. ) ;
#122304=CIRCLE ( 'NONE', #32521, 0.1000000000000000472 ) ;
#122305=FACE_OUTER_BOUND ( 'NONE', #72159, .T. ) ;
#122306=CARTESIAN_POINT ( 'NONE',  ( -11.44999999999999751, 12.50000000000000000, -6.776507416713037024 ) ) ;
#122307=EDGE_CURVE ( 'NONE', #1969, #62361, #81115, .T. ) ;
#122308=ORIENTED_EDGE ( 'NONE', *, *, #80202, .T. ) ;
#122309=DIRECTION ( 'NONE',  ( -0.000000000000000000, 1.000000000000000000, -0.000000000000000000 ) ) ;
#122310=AXIS2_PLACEMENT_3D ( 'NONE', #61443, #109885, #80430 ) ;
#122311=VECTOR ( 'NONE', #39572, 1000.000000000000000 ) ;
#122312=CARTESIAN_POINT ( 'NONE',  ( 14.99999999999989164, 12.50000000000000000, 0.6928203230275494784 ) ) ;
#122313=DIRECTION ( 'NONE',  ( 0.000000000000000000, 1.000000000000000000, 0.000000000000000000 ) ) ;
#122314=ORIENTED_EDGE ( 'NONE', *, *, #55185, .T. ) ;
#122315=CIRCLE ( 'NONE', #116033, 0.1000000000000002554 ) ;
#122316=DIRECTION ( 'NONE',  ( 0.000000000000000000, 0.000000000000000000, 1.000000000000000000 ) ) ;
#122317=DIRECTION ( 'NONE',  ( 0.000000000000000000, -0.000000000000000000, 1.000000000000000000 ) ) ;
#122318=EDGE_LOOP ( 'NONE', ( #110913, #68311, #43842, #111803 ) ) ;
#122320=CIRCLE ( 'NONE', #19814, 0.1000000000000000472 ) ;
#122321=CIRCLE ( 'NONE', #19815, 0.06509327318403745899 ) ;
#122322=ORIENTED_EDGE ( 'NONE', *, *, #19105, .T. ) ;
#122323=ORIENTED_EDGE ( 'NONE', *, *, #105152, .T. ) ;
#122324=ORIENTED_EDGE ( 'NONE', *, *, #60190, .T. ) ;
#122325=CARTESIAN_POINT ( 'NONE',  ( 12.09999999999990550, 2.500000000000000000, 5.022947341949748790 ) ) ;
#122326=VECTOR ( 'NONE', #124879, 1000.000000000000000 ) ;
#122327=CARTESIAN_POINT ( 'NONE',  ( 1.249999999999954259, 2.500000000000000000, -7.188010851410854052 ) ) ;
#122328=CARTESIAN_POINT ( 'NONE',  ( -10.20000000000000462, 2.500000000000000000, -4.676537180435973440 ) ) ;
#122329=AXIS2_PLACEMENT_3D ( 'NONE', #2995, #113591, #15361 ) ;
#122330=DIRECTION ( 'NONE',  ( 0.000000000000000000, 0.000000000000000000, 1.000000000000000000 ) ) ;
#122331=EDGE_LOOP ( 'NONE', ( #59087, #7509, #41990, #97782 ) ) ;
#122332=DIRECTION ( 'NONE',  ( 0.000000000000000000, 0.000000000000000000, 1.000000000000000000 ) ) ;
#122333=VECTOR ( 'NONE', #49532, 1000.000000000000000 ) ;
#122334=EDGE_LOOP ( 'NONE', ( #6310, #18567 ) ) ;
#122335=DIRECTION ( 'NONE',  ( 0.000000000000000000, 0.000000000000000000, -1.000000000000000000 ) ) ;
#122336=CARTESIAN_POINT ( 'NONE',  ( 6.649999999999930189, 2.500000000000000000, -1.572243186433550211 ) ) ;
#122337=DIRECTION ( 'NONE',  ( 0.000000000000000000, 0.000000000000000000, 1.000000000000000000 ) ) ;
#122338=DIRECTION ( 'NONE',  ( 0.000000000000000000, 0.000000000000000000, 1.000000000000000000 ) ) ;
#122339=ORIENTED_EDGE ( 'NONE', *, *, #89048, .F. ) ;
#122340=EDGE_CURVE ( 'NONE', #97064, #69733, #33003, .T. ) ;
#122341=ORIENTED_EDGE ( 'NONE', *, *, #8043, .F. ) ;
#122342=EDGE_LOOP ( 'NONE', ( #80838, #6046, #21942, #56799 ) ) ;
#122343=DIRECTION ( 'NONE',  ( -4.274815082592931898E-19, -0.9999939076577903929, -0.003490651415223739937 ) ) ;
#122344=DIRECTION ( 'NONE',  ( 0.000000000000000000, 0.000000000000000000, 1.000000000000000000 ) ) ;
#122345=FACE_OUTER_BOUND ( 'NONE', #16391, .T. ) ;
#122346=FACE_BOUND ( 'NONE', #37703, .T. ) ;
#122347=DIRECTION ( 'NONE',  ( 0.000000000000000000, 0.000000000000000000, -1.000000000000000000 ) ) ;
#122348=CIRCLE ( 'NONE', #84672, 0.1000000000000002554 ) ;
#122349=DIRECTION ( 'NONE',  ( 0.000000000000000000, -0.000000000000000000, 1.000000000000000000 ) ) ;
#122350=CARTESIAN_POINT ( 'NONE',  ( -1.050000000000038236, 2.500000000000000000, -1.818653347947326138 ) ) ;
#122351=ADVANCED_FACE ( 'NONE', ( #105038 ), #58132, .T. ) ;
#122353=CIRCLE ( 'NONE', #99365, 0.09999999999999982514 ) ;
#122355=FACE_OUTER_BOUND ( 'NONE', #111643, .T. ) ;
#122356=VERTEX_POINT ( 'NONE', #24560 ) ;
#122357=AXIS2_PLACEMENT_3D ( 'NONE', #111589, #23198, #991 ) ;
#122358=VECTOR ( 'NONE', #4312, 1000.000000000000000 ) ;
#122359=FACE_OUTER_BOUND ( 'NONE', #46863, .T. ) ;
#122360=CARTESIAN_POINT ( 'NONE',  ( -7.100000000000017408, 12.50000000000000000, 0.6928203230275494784 ) ) ;
#122361=VERTEX_POINT ( 'NONE', #14716 ) ;
#122362=VERTEX_POINT ( 'NONE', #15360 ) ;
#122363=CARTESIAN_POINT ( 'NONE',  ( 2.899999999999946620, 12.50000000000000000, -3.637306695894650055 ) ) ;
#122364=CARTESIAN_POINT ( 'NONE',  ( 9.199999999999915801, 2.500000000000000000, 4.230127018922196669 ) ) ;
#122365=FACE_BOUND ( 'NONE', #47805, .T. ) ;
#122366=DIRECTION ( 'NONE',  ( 0.000000000000000000, 0.000000000000000000, -1.000000000000000000 ) ) ;
#122367=AXIS2_PLACEMENT_3D ( 'NONE', #2692, #73372, #104135 ) ;
#122368=CIRCLE ( 'NONE', #34643, 0.1000000000000000056 ) ;
#122369=ORIENTED_EDGE ( 'NONE', *, *, #65354, .T. ) ;
#122370=CARTESIAN_POINT ( 'NONE',  ( 21.24754738303297330, 0.7337760880902002292, -4.182111650399407132 ) ) ;
#122371=DIRECTION ( 'NONE',  ( -0.000000000000000000, 1.000000000000000000, -0.000000000000000000 ) ) ;
#122372=ORIENTED_EDGE ( 'NONE', *, *, #50634, .T. ) ;
#122373=CARTESIAN_POINT ( 'NONE',  ( -11.04999999999999893, 2.500000000000000000, 1.718653347947321386 ) ) ;
#122374=DIRECTION ( 'NONE',  ( 0.000000000000000000, 1.000000000000000000, 0.000000000000000000 ) ) ;
#122375=EDGE_CURVE ( 'NONE', #122097, #40089, #129159, .T. ) ;
#122377=VECTOR ( 'NONE', #42721, 1000.000000000000000 ) ;
#122378=ORIENTED_EDGE ( 'NONE', *, *, #126380, .F. ) ;
#122379=CARTESIAN_POINT ( 'NONE',  ( -12.29999999999999538, 2.500000000000000000, 4.676537180435972552 ) ) ;
#122380=FACE_OUTER_BOUND ( 'NONE', #12813, .T. ) ;
#122381=EDGE_CURVE ( 'NONE', #63670, #126127, #28889, .T. ) ;
#122382=ORIENTED_EDGE ( 'NONE', *, *, #62386, .F. ) ;
#122383=CARTESIAN_POINT ( 'NONE',  ( -12.04999999999999716, 2.500000000000000000, -2.165063509461097713 ) ) ;
#122385=DIRECTION ( 'NONE',  ( 0.000000000000000000, 1.000000000000000000, 0.000000000000000000 ) ) ;
#122386=ORIENTED_EDGE ( 'NONE', *, *, #46646, .T. ) ;
#122387=EDGE_CURVE ( 'NONE', #110101, #26341, #53915, .T. ) ;
#122388=ORIENTED_EDGE ( 'NONE', *, *, #51996, .T. ) ;
#122389=ADVANCED_FACE ( 'NONE', ( #50026 ), #49378, .T. ) ;
#122390=DIRECTION ( 'NONE',  ( 0.000000000000000000, 1.000000000000000000, 0.000000000000000000 ) ) ;
#122391=CIRCLE ( 'NONE', #97336, 0.06509327318403745899 ) ;
#122392=VERTEX_POINT ( 'NONE', #77520 ) ;
#122393=DIRECTION ( 'NONE',  ( -0.000000000000000000, 1.000000000000000000, -0.000000000000000000 ) ) ;
#122394=LINE ( 'NONE', #53643, #13865 ) ;
#122395=DIRECTION ( 'NONE',  ( 0.000000000000000000, 0.000000000000000000, -1.000000000000000000 ) ) ;
#122396=VERTEX_POINT ( 'NONE', #87964 ) ;
#122397=ADVANCED_FACE ( 'NONE', ( #7487 ), #91567, .T. ) ;
#122398=CIRCLE ( 'NONE', #84813, 0.06509327318403745899 ) ;
#122399=CARTESIAN_POINT ( 'NONE',  ( 7.099999999999926814, 2.500000000000000000, -2.276824562219559311E-15 ) ) ;
#122400=DIRECTION ( 'NONE',  ( 0.000000000000000000, 0.000000000000000000, 1.000000000000000000 ) ) ;
#122401=DIRECTION ( 'NONE',  ( 0.000000000000000000, 0.000000000000000000, -1.000000000000000000 ) ) ;
#122402=PLANE ( 'NONE',  #8928 ) ;
#122403=EDGE_CURVE ( 'NONE', #2627, #12624, #68990, .T. ) ;
#122404=DIRECTION ( 'NONE',  ( 0.000000000000000000, 0.000000000000000000, 1.000000000000000000 ) ) ;
#122405=AXIS2_PLACEMENT_3D ( 'NONE', #59003, #85861, #57722 ) ;
#122406=ORIENTED_EDGE ( 'NONE', *, *, #67483, .F. ) ;
#122407=ORIENTED_EDGE ( 'NONE', *, *, #1690, .T. ) ;
#122408=AXIS2_PLACEMENT_3D ( 'NONE', #77359, #71231, #78660 ) ;
#122409=CARTESIAN_POINT ( 'NONE',  ( 10.19999999999991047, 2.500000000000000000, -3.983716857408426293 ) ) ;
#122410=ORIENTED_EDGE ( 'NONE', *, *, #36108, .F. ) ;
#122411=CARTESIAN_POINT ( 'NONE',  ( 4.599999999999940137, 12.50000000000000000, -5.088040615133791356 ) ) ;
#122412=ORIENTED_EDGE ( 'NONE', *, *, #38193, .T. ) ;
#122413=EDGE_LOOP ( 'NONE', ( #15483, #16078, #17610, #56034 ) ) ;
#122414=EDGE_LOOP ( 'NONE', ( #53000, #105085, #42891, #16271 ) ) ;
#122415=CARTESIAN_POINT ( 'NONE',  ( 2.099999999999950351, 2.500000000000000000, -5.122947341949753763 ) ) ;
#122416=AXIS2_PLACEMENT_3D ( 'NONE', #42119, #89918, #41500 ) ;
#122417=DIRECTION ( 'NONE',  ( 0.000000000000000000, -0.9999939076577903929, 0.003490651415223739937 ) ) ;
#122418=CIRCLE ( 'NONE', #38816, 0.1000000000000002554 ) ;
#122419=DIRECTION ( 'NONE',  ( -0.000000000000000000, 1.000000000000000000, -0.000000000000000000 ) ) ;
#122420=CONICAL_SURFACE ( 'NONE', #128704, 0.1000000000000002554, 0.003490658503988666988 ) ;
#122421=PLANE ( 'NONE',  #13913 ) ;
#122422=DIRECTION ( 'NONE',  ( -4.274815082592931898E-19, -0.9999939076577903929, -0.003490651415223739937 ) ) ;
#122423=PLANE ( 'NONE',  #105067 ) ;
#122424=CONICAL_SURFACE ( 'NONE', #84762, 0.1000000000000002554, 0.003490658503988666988 ) ;
#122425=LINE ( 'NONE', #30834, #30932 ) ;
#122426=CARTESIAN_POINT ( 'NONE',  ( -2.050000000000033129, 12.50000000000000000, 6.560283801567334372 ) ) ;
#122427=DIRECTION ( 'NONE',  ( -0.000000000000000000, -1.000000000000000000, -0.000000000000000000 ) ) ;
#122428=EDGE_LOOP ( 'NONE', ( #86571, #92362, #60899, #62307 ) ) ;
#122429=EDGE_CURVE ( 'NONE', #17323, #103868, #62245, .T. ) ;
#122430=FACE_OUTER_BOUND ( 'NONE', #48235, .T. ) ;
#122431=EDGE_LOOP ( 'NONE', ( #4893, #21361 ) ) ;
#122432=VERTEX_POINT ( 'NONE', #108899 ) ;
#122433=CARTESIAN_POINT ( 'NONE',  ( 8.949999999999921130, 12.50000000000000000, 1.818653347947321475 ) ) ;
#122434=CARTESIAN_POINT ( 'NONE',  ( -9.350000000000008527, 2.500000000000000000, -6.841600689897072485 ) ) ;
#122435=AXIS2_PLACEMENT_3D ( 'NONE', #13202, #103544, #3398 ) ;
#122436=DIRECTION ( 'NONE',  ( 0.000000000000000000, 1.000000000000000000, 0.000000000000000000 ) ) ;
#122437=EDGE_CURVE ( 'NONE', #90797, #15482, #24675, .T. ) ;
#122439=CARTESIAN_POINT ( 'NONE',  ( -4.200000000000029488, 2.500000000000000000, -4.330127018922201643 ) ) ;
#122440=DIRECTION ( 'NONE',  ( 0.000000000000000000, 1.000000000000000000, 0.000000000000000000 ) ) ;
#122441=FACE_OUTER_BOUND ( 'NONE', #121998, .T. ) ;
#122442=EDGE_LOOP ( 'NONE', ( #18400, #94713 ) ) ;
#122443=ADVANCED_FACE ( 'NONE', ( #97805 ), #62334, .T. ) ;
#122444=AXIS2_PLACEMENT_3D ( 'NONE', #7902, #17716, #38691 ) ;
#122445=ADVANCED_FACE ( 'NONE', ( #27770 ), #67695, .T. ) ;
#122446=CIRCLE ( 'NONE', #55543, 0.06509327318403745899 ) ;
#122447=EDGE_CURVE ( 'NONE', #81045, #66966, #74848, .T. ) ;
#122448=AXIS2_PLACEMENT_3D ( 'NONE', #110909, #60561, #23178 ) ;
#122449=VERTEX_POINT ( 'NONE', #28436 ) ;
#122450=EDGE_LOOP ( 'NONE', ( #88528, #63270 ) ) ;
#122451=AXIS2_PLACEMENT_3D ( 'NONE', #786, #51838, #69528 ) ;
#122452=EDGE_CURVE ( 'NONE', #38135, #20260, #127090, .T. ) ;
#122453=ORIENTED_EDGE ( 'NONE', *, *, #80935, .T. ) ;
#122454=ORIENTED_EDGE ( 'NONE', *, *, #34235, .T. ) ;
#122455=CARTESIAN_POINT ( 'NONE',  ( 4.199999999999938005, 12.50000000000000000, 4.395220292106234439 ) ) ;
#122456=DIRECTION ( 'NONE',  ( -0.000000000000000000, 1.000000000000000000, -0.000000000000000000 ) ) ;
#122457=ADVANCED_FACE ( 'NONE', ( #67036 ), #64370, .T. ) ;
#122458=AXIS2_PLACEMENT_3D ( 'NONE', #40579, #83704, #3215 ) ;
#122459=ADVANCED_FACE ( 'NONE', ( #48725 ), #66426, .T. ) ;
#122460=CARTESIAN_POINT ( 'NONE',  ( 6.049999999999932321, 12.50000000000000000, 6.841600689897072485 ) ) ;
#122461=DIRECTION ( 'NONE',  ( 0.000000000000000000, 0.000000000000000000, 1.000000000000000000 ) ) ;
#122462=AXIS2_PLACEMENT_3D ( 'NONE', #128380, #111260, #38717 ) ;
#122463=CIRCLE ( 'NONE', #114127, 0.06509327318403745899 ) ;
#122464=CARTESIAN_POINT ( 'NONE',  ( 9.349999999999919709, 2.500000000000000000, 1.818653347947321475 ) ) ;
#122465=EDGE_LOOP ( 'NONE', ( #124231, #13548, #64099, #38898 ) ) ;
#122466=DIRECTION ( 'NONE',  ( -0.000000000000000000, 1.000000000000000000, -0.000000000000000000 ) ) ;
#122467=DIRECTION ( 'NONE',  ( 0.000000000000000000, 0.000000000000000000, -1.000000000000000000 ) ) ;
#122468=CARTESIAN_POINT ( 'NONE',  ( 5.849999999999935696, 2.500000000000000000, -6.595190528383302109 ) ) ;
#122469=CARTESIAN_POINT ( 'NONE',  ( 0.6499999999999561684, 2.500000000000000000, -1.818653347947325916 ) ) ;
#122470=EDGE_LOOP ( 'NONE', ( #83922, #94149, #23994, #71916 ) ) ;
#122471=CONICAL_SURFACE ( 'NONE', #51374, 0.1000000000000002554, 0.003490658503988666988 ) ;
#122472=AXIS2_PLACEMENT_3D ( 'NONE', #13863, #53795, #54435 ) ;
#122473=VERTEX_POINT ( 'NONE', #8130 ) ;
#122474=VERTEX_POINT ( 'NONE', #17956 ) ;
#122475=DIRECTION ( 'NONE',  ( 0.000000000000000000, 0.000000000000000000, 1.000000000000000000 ) ) ;
#122476=ORIENTED_EDGE ( 'NONE', *, *, #117738, .F. ) ;
#122477=CARTESIAN_POINT ( 'NONE',  ( -1.050000000000037792, 2.500000000000000000, 6.148780366869520009 ) ) ;
#122478=DIRECTION ( 'NONE',  ( -4.274815082592931898E-19, -0.9999939076577903929, -0.003490651415223739937 ) ) ;
#122479=EDGE_LOOP ( 'NONE', ( #23203, #118920, #60618, #25765 ) ) ;
#122480=CARTESIAN_POINT ( 'NONE',  ( -13.29999999999999005, 2.500000000000000000, 1.843143693225357538E-15 ) ) ;
#122481=DIRECTION ( 'NONE',  ( 0.000000000000000000, -0.9999939076577903929, 0.003490651415223739937 ) ) ;
#122482=ADVANCED_FACE ( 'NONE', ( #29714 ), #69638, .T. ) ;
#122483=CARTESIAN_POINT ( 'NONE',  ( 1.449999999999951328, 2.500000000000000000, 2.511473670974873507 ) ) ;
#122484=DIRECTION ( 'NONE',  ( 0.000000000000000000, -0.9999939076577903929, 0.003490651415223739937 ) ) ;
#122485=VECTOR ( 'NONE', #114170, 1000.000000000000000 ) ;
#122486=CARTESIAN_POINT ( 'NONE',  ( -11.25000000000000178, 12.50000000000000000, -1.407149913249508666 ) ) ;
#122487=AXIS2_PLACEMENT_3D ( 'NONE', #18454, #48567, #39413 ) ;
#122488=VERTEX_POINT ( 'NONE', #57242 ) ;
#122489=EDGE_LOOP ( 'NONE', ( #104590, #17969, #2780, #15439 ) ) ;
#122490=DIRECTION ( 'NONE',  ( 0.000000000000000000, 1.000000000000000000, 0.000000000000000000 ) ) ;
#122491=FACE_OUTER_BOUND ( 'NONE', #40681, .T. ) ;
#122492=FACE_OUTER_BOUND ( 'NONE', #37954, .T. ) ;
#122493=LINE ( 'NONE', #120554, #104405 ) ;
#122494=EDGE_CURVE ( 'NONE', #8018, #35473, #5770, .T. ) ;
#122495=ORIENTED_EDGE ( 'NONE', *, *, #12712, .F. ) ;
#122496=VERTEX_POINT ( 'NONE', #12003 ) ;
#122497=LINE ( 'NONE', #42665, #106501 ) ;
#122498=FACE_OUTER_BOUND ( 'NONE', #4425, .T. ) ;
#122499=DIRECTION ( 'NONE',  ( 0.000000000000000000, 0.000000000000000000, 1.000000000000000000 ) ) ;
#122500=CARTESIAN_POINT ( 'NONE',  ( -2.050000000000032685, 2.500000000000000000, -2.165063509461101710 ) ) ;
#122501=EDGE_LOOP ( 'NONE', ( #29818, #75415 ) ) ;
#122502=AXIS2_PLACEMENT_3D ( 'NONE', #56433, #85260, #6659 ) ;
#122503=CARTESIAN_POINT ( 'NONE',  ( -12.29999999999999538, 2.500000000000000000, -4.676537180435976104 ) ) ;
#122505=CARTESIAN_POINT ( 'NONE',  ( -13.29999999999999005, 2.500000000000000000, 1.843143693225357538E-15 ) ) ;
#122506=CIRCLE ( 'NONE', #111754, 0.06509327318403745899 ) ;
#122507=ORIENTED_EDGE ( 'NONE', *, *, #13977, .F. ) ;
#122508=DIRECTION ( 'NONE',  ( 0.000000000000000000, 0.000000000000000000, 1.000000000000000000 ) ) ;
#122509=ORIENTED_EDGE ( 'NONE', *, *, #58136, .T. ) ;
#122510=DIRECTION ( 'NONE',  ( 0.000000000000000000, 1.000000000000000000, 0.000000000000000000 ) ) ;
#122511=ORIENTED_EDGE ( 'NONE', *, *, #37934, .T. ) ;
#122512=FACE_OUTER_BOUND ( 'NONE', #21567, .T. ) ;
#122513=LINE ( 'NONE', #112696, #43909 ) ;
#122514=ORIENTED_EDGE ( 'NONE', *, *, #5425, .F. ) ;
#122515=EDGE_LOOP ( 'NONE', ( #89364, #49927, #104409, #66220 ) ) ;
#122516=DIRECTION ( 'NONE',  ( 0.000000000000000000, 0.000000000000000000, -1.000000000000000000 ) ) ;
#122517=CARTESIAN_POINT ( 'NONE',  ( -7.900000000000014566, 12.50000000000000000, -0.6928203230275541413 ) ) ;
#122518=AXIS2_PLACEMENT_3D ( 'NONE', #12409, #52343, #73270 ) ;
#122521=DIRECTION ( 'NONE',  ( -0.000000000000000000, -1.000000000000000000, -0.000000000000000000 ) ) ;
#122522=CIRCLE ( 'NONE', #127021, 0.06509327318403745899 ) ;
#122523=DIRECTION ( 'NONE',  ( 0.000000000000000000, -0.9999939076577903929, 0.003490651415223739937 ) ) ;
#122524=DIRECTION ( 'NONE',  ( 0.000000000000000000, -0.9999939076577903929, 0.003490651415223739937 ) ) ;
#122525=CARTESIAN_POINT ( 'NONE',  ( -0.4000000000000404898, 2.500000000000000000, 5.022947341949748790 ) ) ;
#122526=CONICAL_SURFACE ( 'NONE', #112158, 0.1000000000000000472, 0.003490658503988666988 ) ;
#122528=AXIS2_PLACEMENT_3D ( 'NONE', #123789, #55069, #43331 ) ;
#122529=EDGE_CURVE ( 'NONE', #102213, #105669, #23114, .T. ) ;
#122530=VERTEX_POINT ( 'NONE', #80760 ) ;
#122531=AXIS2_PLACEMENT_3D ( 'NONE', #4006, #68085, #16384 ) ;
#122532=ORIENTED_EDGE ( 'NONE', *, *, #58465, .T. ) ;
#122533=CARTESIAN_POINT ( 'NONE',  ( -1.650000000000034772, 12.50000000000000000, 6.495190528383297135 ) ) ;
#122534=ORIENTED_EDGE ( 'NONE', *, *, #92235, .T. ) ;
#122535=CARTESIAN_POINT ( 'NONE',  ( 9.199999999999919353, 12.50000000000000000, -2.276824562219559311E-15 ) ) ;
#122536=CARTESIAN_POINT ( 'NONE',  ( -7.500000000000011546, 12.50000000000000000, 3.637306695894644726 ) ) ;
#122537=LINE ( 'NONE', #72154, #30174 ) ;
#122538=EDGE_LOOP ( 'NONE', ( #90981, #25116 ) ) ;
#122539=VERTEX_POINT ( 'NONE', #30381 ) ;
#122540=EDGE_CURVE ( 'NONE', #91908, #123357, #120680, .T. ) ;
#122541=FACE_BOUND ( 'NONE', #37878, .T. ) ;
#122542=ORIENTED_EDGE ( 'NONE', *, *, #128169, .F. ) ;
#122543=ADVANCED_FACE ( 'NONE', ( #101684 ), #40188, .T. ) ;
#122544=FACE_OUTER_BOUND ( 'NONE', #86014, .T. ) ;
#122545=CARTESIAN_POINT ( 'NONE',  ( 19.01901804971378240, -2.576149587736908941, 2.431039412660930044 ) ) ;
#122546=VECTOR ( 'NONE', #121677, 1000.000000000000000 ) ;
#122547=LINE ( 'NONE', #71499, #109894 ) ;
#122548=FACE_OUTER_BOUND ( 'NONE', #45681, .T. ) ;
#122550=CIRCLE ( 'NONE', #28551, 0.06509327318403743123 ) ;
#122551=AXIS2_PLACEMENT_3D ( 'NONE', #9853, #20321, #110625 ) ;
#122552=CARTESIAN_POINT ( 'NONE',  ( 15.19999999999989271, 12.50000000000000000, -0.3464101615137783474 ) ) ;
#122553=EDGE_CURVE ( 'NONE', #30037, #72858, #43467, .T. ) ;
#122554=DIRECTION ( 'NONE',  ( 0.000000000000000000, 1.000000000000000000, 0.000000000000000000 ) ) ;
#122555=ADVANCED_FACE ( 'NONE', ( #82028 ), #3734, .T. ) ;
#122556=CARTESIAN_POINT ( 'NONE',  ( 9.349999999999919709, 2.500000000000000000, -6.248780366869526759 ) ) ;
#122557=FACE_OUTER_BOUND ( 'NONE', #125517, .T. ) ;
#122558=CARTESIAN_POINT ( 'NONE',  ( -6.900000000000019007, 2.500000000000000000, 0.3464101615137735735 ) ) ;
#122559=EDGE_CURVE ( 'NONE', #67957, #29548, #93628, .T. ) ;
#122560=DIRECTION ( 'NONE',  ( 0.000000000000000000, 0.000000000000000000, 1.000000000000000000 ) ) ;
#122561=ORIENTED_EDGE ( 'NONE', *, *, #79815, .T. ) ;
#122562=ORIENTED_EDGE ( 'NONE', *, *, #29898, .F. ) ;
#122563=EDGE_LOOP ( 'NONE', ( #44482, #16132, #114085, #95381 ) ) ;
#122564=DIRECTION ( 'NONE',  ( -0.000000000000000000, 1.000000000000000000, -0.000000000000000000 ) ) ;
#122565=ORIENTED_EDGE ( 'NONE', *, *, #67463, .F. ) ;
#122566=DIRECTION ( 'NONE',  ( 0.000000000000000000, 0.000000000000000000, -1.000000000000000000 ) ) ;
#122567=ORIENTED_EDGE ( 'NONE', *, *, #648, .F. ) ;
#122568=ORIENTED_EDGE ( 'NONE', *, *, #110666, .T. ) ;
#122569=VERTEX_POINT ( 'NONE', #72866 ) ;
#122570=FACE_OUTER_BOUND ( 'NONE', #17580, .T. ) ;
#122571=CARTESIAN_POINT ( 'NONE',  ( 1.249999999999988898, 2.500000000000000000, -6.495190528383302464 ) ) ;
#122572=DIRECTION ( 'NONE',  ( 0.000000000000000000, 0.000000000000000000, 1.000000000000000000 ) ) ;
#122573=CARTESIAN_POINT ( 'NONE',  ( -0.8500000000000386136, 12.50000000000000000, 2.857883832488649301 ) ) ;
#122574=DIRECTION ( 'NONE',  ( -0.000000000000000000, 1.000000000000000000, -0.000000000000000000 ) ) ;
#122575=CARTESIAN_POINT ( 'NONE',  ( 5.649999999999934630, 2.500000000000000000, 6.741600689897071952 ) ) ;
#122576=VERTEX_POINT ( 'NONE', #31034 ) ;
#122577=CARTESIAN_POINT ( 'NONE',  ( 1.649999999999951950, 2.500000000000000000, -5.802370205355749988 ) ) ;
#122578=ORIENTED_EDGE ( 'NONE', *, *, #2875, .F. ) ;
#122579=ORIENTED_EDGE ( 'NONE', *, *, #74952, .T. ) ;
#122580=EDGE_LOOP ( 'NONE', ( #50008, #79228, #71177, #29033 ) ) ;
#122581=CIRCLE ( 'NONE', #24377, 0.06509327318403745899 ) ;
#122583=ORIENTED_EDGE ( 'NONE', *, *, #103226, .T. ) ;
#122584=ORIENTED_EDGE ( 'NONE', *, *, #81655, .T. ) ;
#122585=ORIENTED_EDGE ( 'NONE', *, *, #25008, .F. ) ;
#122586=DIRECTION ( 'NONE',  ( 0.000000000000000000, 1.000000000000000000, 0.000000000000000000 ) ) ;
#122587=CIRCLE ( 'NONE', #11845, 0.09999999999999982514 ) ;
#122588=DIRECTION ( 'NONE',  ( 0.000000000000000000, -0.000000000000000000, 1.000000000000000000 ) ) ;
#122589=CARTESIAN_POINT ( 'NONE',  ( 14.79999999999989413, 2.500000000000000000, -0.2464101615137782308 ) ) ;
#122590=DIRECTION ( 'NONE',  ( 0.000000000000000000, 0.000000000000000000, 1.000000000000000000 ) ) ;
#122591=FACE_OUTER_BOUND ( 'NONE', #29125, .T. ) ;
#122592=ADVANCED_FACE ( 'NONE', ( #62415 ), #120816, .T. ) ;
#122593=CARTESIAN_POINT ( 'NONE',  ( 1.849999999999949685, 2.500000000000000000, 1.718653347947321386 ) ) ;
#122594=ADVANCED_FACE ( 'NONE', ( #112148 ), #78975, .T. ) ;
#122595=EDGE_CURVE ( 'NONE', #123681, #8315, #91864, .T. ) ;
#122596=CARTESIAN_POINT ( 'NONE',  ( 9.149999999999920419, 12.50000000000000000, 2.857883832488649301 ) ) ;
#122597=CONICAL_SURFACE ( 'NONE', #28507, 0.1000000000000002554, 0.003490658503988666988 ) ;
#122598=CIRCLE ( 'NONE', #22258, 0.1000000000000000056 ) ;
#122599=ORIENTED_EDGE ( 'NONE', *, *, #40895, .F. ) ;
#122600=PLANE ( 'NONE',  #102807 ) ;
#122601=ORIENTED_EDGE ( 'NONE', *, *, #21943, .F. ) ;
#122602=ADVANCED_FACE ( 'NONE', ( #12639 ), #39279, .T. ) ;
#122604=DIRECTION ( 'NONE',  ( -0.000000000000000000, -1.000000000000000000, -0.000000000000000000 ) ) ;
#122605=EDGE_CURVE ( 'NONE', #2437, #28355, #95693, .T. ) ;
#122606=ORIENTED_EDGE ( 'NONE', *, *, #90346, .F. ) ;
#122607=EDGE_CURVE ( 'NONE', #45548, #14446, #100394, .T. ) ;
#122608=CARTESIAN_POINT ( 'NONE',  ( 9.399999999999915090, 2.500000000000000000, 4.676537180435972552 ) ) ;
#122609=EDGE_CURVE ( 'NONE', #89145, #702, #43564, .T. ) ;
#122610=EDGE_CURVE ( 'NONE', #43078, #8727, #93714, .T. ) ;
#122611=CARTESIAN_POINT ( 'NONE',  ( 11.04999999999991012, 2.500000000000000000, 6.941600689897073018 ) ) ;
#122612=VERTEX_POINT ( 'NONE', #53235 ) ;
#122613=ORIENTED_EDGE ( 'NONE', *, *, #121073, .F. ) ;
#122614=CARTESIAN_POINT ( 'NONE',  ( 3.549999999999942091, 2.500000000000000000, 2.511473670974873507 ) ) ;
#122615=CARTESIAN_POINT ( 'NONE',  ( -8.350000000000013856, 12.50000000000000000, -7.253104124594885960 ) ) ;
#122616=DIRECTION ( 'NONE',  ( -0.000000000000000000, 1.000000000000000000, -0.000000000000000000 ) ) ;
#122617=CIRCLE ( 'NONE', #34799, 0.06509327318403745899 ) ;
#122618=DIRECTION ( 'NONE',  ( 0.000000000000000000, 1.000000000000000000, 0.000000000000000000 ) ) ;
#122619=ADVANCED_FACE ( 'NONE', ( #13280 ), #87444, .T. ) ;
#122620=LINE ( 'NONE', #23120, #81449 ) ;
#122621=VERTEX_POINT ( 'NONE', #41499 ) ;
#122622=FACE_OUTER_BOUND ( 'NONE', #61995, .T. ) ;
#122623=AXIS2_PLACEMENT_3D ( 'NONE', #499, #61382, #101308 ) ;
#122624=AXIS2_PLACEMENT_3D ( 'NONE', #43966, #34145, #100930 ) ;
#122625=EDGE_LOOP ( 'NONE', ( #62932, #110932 ) ) ;
#122626=CARTESIAN_POINT ( 'NONE',  ( 12.89999999999989910, 2.500000000000000000, -0.7928203230275543412 ) ) ;
#122627=DIRECTION ( 'NONE',  ( 0.000000000000000000, 0.000000000000000000, -1.000000000000000000 ) ) ;
#122628=AXIS2_PLACEMENT_3D ( 'NONE', #63434, #113830, #64076 ) ;
#122630=FACE_OUTER_BOUND ( 'NONE', #99292, .T. ) ;
#122631=LINE ( 'NONE', #32977, #69545 ) ;
#122632=CARTESIAN_POINT ( 'NONE',  ( -10.40000000000000213, 2.500000000000000000, -0.1000000000000022815 ) ) ;
#122633=CARTESIAN_POINT ( 'NONE',  ( -11.64999999999999858, 2.500000000000000000, -1.572243186433546214 ) ) ;
#122634=ORIENTED_EDGE ( 'NONE', *, *, #84894, .T. ) ;
#122635=CIRCLE ( 'NONE', #36961, 0.1000000000000002554 ) ;
#122636=DIRECTION ( 'NONE',  ( 0.000000000000000000, 1.000000000000000000, 0.000000000000000000 ) ) ;
#122637=VECTOR ( 'NONE', #94709, 1000.000000000000000 ) ;
#122638=CARTESIAN_POINT ( 'NONE',  ( 7.049999999999928768, 12.50000000000000000, 6.495190528383297135 ) ) ;
#122639=CARTESIAN_POINT ( 'NONE',  ( 0.5999999999999560130, 12.50000000000000000, -3.983716857408426293 ) ) ;
#122640=ORIENTED_EDGE ( 'NONE', *, *, #81120, .T. ) ;
#122641=DIRECTION ( 'NONE',  ( 0.000000000000000000, 0.000000000000000000, -1.000000000000000000 ) ) ;
#122643=ORIENTED_EDGE ( 'NONE', *, *, #126383, .T. ) ;
#122644=ORIENTED_EDGE ( 'NONE', *, *, #70517, .F. ) ;
#122645=CARTESIAN_POINT ( 'NONE',  ( 2.049999999999950084, 2.500000000000000000, 2.265063509461097357 ) ) ;
#122646=ORIENTED_EDGE ( 'NONE', *, *, #46130, .F. ) ;
#122647=CARTESIAN_POINT ( 'NONE',  ( 12.04999999999990834, 12.50000000000000000, -2.165063509461101710 ) ) ;
#122648=CARTESIAN_POINT ( 'NONE',  ( 13.34999999999990017, 2.500000000000000000, 2.857883832488649301 ) ) ;
#122649=DIRECTION ( 'NONE',  ( -0.000000000000000000, 1.000000000000000000, -0.000000000000000000 ) ) ;
#122650=ORIENTED_EDGE ( 'NONE', *, *, #24422, .F. ) ;
#122651=CARTESIAN_POINT ( 'NONE',  ( -9.150000000000009237, 2.500000000000000000, 2.165063509461097713 ) ) ;
#122652=CARTESIAN_POINT ( 'NONE',  ( -4.250072516143177381E-14, 2.500000000000000000, -3.637306695894650055 ) ) ;
#122653=EDGE_CURVE ( 'NONE', #18590, #69752, #76993, .T. ) ;
#122654=EDGE_LOOP ( 'NONE', ( #26821, #44778, #74643, #36279 ) ) ;
#122655=VECTOR ( 'NONE', #68776, 1000.000000000000000 ) ;
#122656=ORIENTED_EDGE ( 'NONE', *, *, #62119, .T. ) ;
#122657=CONICAL_SURFACE ( 'NONE', #68367, 0.09999999999999982514, 0.003490658503988666988 ) ;
#122658=VERTEX_POINT ( 'NONE', #13927 ) ;
#122659=DIRECTION ( 'NONE',  ( 0.000000000000000000, 0.000000000000000000, 1.000000000000000000 ) ) ;
#122660=FACE_OUTER_BOUND ( 'NONE', #82290, .T. ) ;
#122661=FACE_OUTER_BOUND ( 'NONE', #62395, .T. ) ;
#122662=ORIENTED_EDGE ( 'NONE', *, *, #67077, .T. ) ;
#122663=CARTESIAN_POINT ( 'NONE',  ( 11.64999999999990443, 12.50000000000000000, -5.802370205355749988 ) ) ;
#122664=DIRECTION ( 'NONE',  ( 0.000000000000000000, 0.000000000000000000, -1.000000000000000000 ) ) ;
#122665=ORIENTED_EDGE ( 'NONE', *, *, #83606, .T. ) ;
#122666=CONICAL_SURFACE ( 'NONE', #64173, 0.1000000000000000472, 0.003490658503988666988 ) ;
#122667=CIRCLE ( 'NONE', #26525, 0.1000000000000002554 ) ;
#122668=CARTESIAN_POINT ( 'NONE',  ( 7.899999999999921307, 12.50000000000000000, -2.385244779468109755E-15 ) ) ;
#122669=CARTESIAN_POINT ( 'NONE',  ( 3.099999999999945466, 2.500000000000000000, -3.883716857408426648 ) ) ;
#122670=FACE_OUTER_BOUND ( 'NONE', #89958, .T. ) ;
#122671=CARTESIAN_POINT ( 'NONE',  ( -11.89999999999999503, 2.500000000000000000, 4.083716857408420609 ) ) ;
#122672=DIRECTION ( 'NONE',  ( -0.000000000000000000, -1.000000000000000000, -0.000000000000000000 ) ) ;
#122673=AXIS2_PLACEMENT_3D ( 'NONE', #5973, #64898, #4673 ) ;
#122674=CARTESIAN_POINT ( 'NONE',  ( 11.84999999999990372, 12.50000000000000000, -6.776507416713040577 ) ) ;
#122675=CARTESIAN_POINT ( 'NONE',  ( 1.649999999999951950, 2.500000000000000000, -5.702370205355749455 ) ) ;
#122676=AXIS2_PLACEMENT_3D ( 'NONE', #59025, #100865, #21682 ) ;
#122677=CIRCLE ( 'NONE', #126888, 0.1000000000000002554 ) ;
#122678=CIRCLE ( 'NONE', #11857, 0.1000000000000002554 ) ;
#122679=ADVANCED_FACE ( 'NONE', ( #44049 ), #5957, .T. ) ;
#122680=VERTEX_POINT ( 'NONE', #5402 ) ;
#122681=ORIENTED_EDGE ( 'NONE', *, *, #92064, .F. ) ;
#122682=ORIENTED_EDGE ( 'NONE', *, *, #39830, .T. ) ;
#122683=ORIENTED_EDGE ( 'NONE', *, *, #12046, .T. ) ;
#122684=FACE_OUTER_BOUND ( 'NONE', #99007, .T. ) ;
#122686=LINE ( 'NONE', #61192, #122008 ) ;
#122687=ORIENTED_EDGE ( 'NONE', *, *, #1956, .F. ) ;
#122688=FACE_BOUND ( 'NONE', #76778, .T. ) ;
#122689=ADVANCED_FACE ( 'NONE', ( #16498 ), #39370, .T. ) ;
#122690=DIRECTION ( 'NONE',  ( 0.000000000000000000, 1.000000000000000000, 0.000000000000000000 ) ) ;
#122691=DIRECTION ( 'NONE',  ( 0.000000000000000000, 0.000000000000000000, 1.000000000000000000 ) ) ;
#122692=CARTESIAN_POINT ( 'NONE',  ( -9.350000000000006750, 2.500000000000000000, 2.411473670974873862 ) ) ;
#122693=DIRECTION ( 'NONE',  ( -4.274815082592931898E-19, -0.9999939076577903929, -0.003490651415223739937 ) ) ;
#122694=CARTESIAN_POINT ( 'NONE',  ( -8.750000000000008882, 12.50000000000000000, -2.857883832488653741 ) ) ;
#122695=EDGE_CURVE ( 'NONE', #105744, #63695, #125189, .T. ) ;
#122696=DIRECTION ( 'NONE',  ( -0.000000000000000000, -1.000000000000000000, -0.000000000000000000 ) ) ;
#122697=EDGE_CURVE ( 'NONE', #23087, #949, #26350, .T. ) ;
#122698=DIRECTION ( 'NONE',  ( 0.000000000000000000, 1.000000000000000000, 0.000000000000000000 ) ) ;
#122699=CARTESIAN_POINT ( 'NONE',  ( -2.499999999999996003, 12.50000000000000000, -4.330127018922201643 ) ) ;
#122700=EDGE_CURVE ( 'NONE', #113873, #42980, #34893, .T. ) ;
#122701=CARTESIAN_POINT ( 'NONE',  ( 1.449999999999949551, 2.500000000000000000, 6.841600689897072485 ) ) ;
#122702=ADVANCED_FACE ( 'NONE', ( #73492 ), #68670, .T. ) ;
#122703=VECTOR ( 'NONE', #114962, 1000.000000000000000 ) ;
#122704=EDGE_CURVE ( 'NONE', #13568, #75204, #47755, .T. ) ;
#122705=VERTEX_POINT ( 'NONE', #94421 ) ;
#122706=ORIENTED_EDGE ( 'NONE', *, *, #64494, .T. ) ;
#122707=CIRCLE ( 'NONE', #34993, 0.09999999999999982514 ) ;
#122708=ORIENTED_EDGE ( 'NONE', *, *, #5042, .T. ) ;
#122709=ORIENTED_EDGE ( 'NONE', *, *, #97151, .F. ) ;
#122710=ORIENTED_EDGE ( 'NONE', *, *, #6971, .T. ) ;
#122711=ORIENTED_EDGE ( 'NONE', *, *, #49604, .T. ) ;
#122712=DIRECTION ( 'NONE',  ( 0.000000000000000000, -0.9999939076577903929, 0.003490651415223739937 ) ) ;
#122713=EDGE_LOOP ( 'NONE', ( #77946, #11774 ) ) ;
#122714=ADVANCED_FACE ( 'NONE', ( #34249 ), #114078, .T. ) ;
#122715=AXIS2_PLACEMENT_3D ( 'NONE', #80361, #109810, #1770 ) ;
#122716=EDGE_LOOP ( 'NONE', ( #91361, #12226 ) ) ;
#122717=CIRCLE ( 'NONE', #1516, 0.06509327318403745899 ) ;
#122718=EDGE_CURVE ( 'NONE', #126712, #112141, #5868, .T. ) ;
#122719=CARTESIAN_POINT ( 'NONE',  ( 16.04744068708433247, -2.499999999999937828, 6.586254740843006772 ) ) ;
#122721=CARTESIAN_POINT ( 'NONE',  ( -10.65000000000000213, 12.50000000000000000, 2.511473670974873507 ) ) ;
#122722=CONICAL_SURFACE ( 'NONE', #66279, 0.1000000000000002554, 0.003490658503988666988 ) ;
#122723=ORIENTED_EDGE ( 'NONE', *, *, #27902, .F. ) ;
#122724=CARTESIAN_POINT ( 'NONE',  ( 7.049999999999928768, 2.500000000000000000, -2.065063509461102065 ) ) ;
#122725=VECTOR ( 'NONE', #41383, 1000.000000000000000 ) ;
#122726=EDGE_LOOP ( 'NONE', ( #28493, #29687, #70152, #42713 ) ) ;
#122727=CONICAL_SURFACE ( 'NONE', #18260, 0.1000000000000002554, 0.003490658503988666988 ) ;
#122728=AXIS2_PLACEMENT_3D ( 'NONE', #74571, #15631, #66034 ) ;
#122729=EDGE_LOOP ( 'NONE', ( #69181, #117046 ) ) ;
#122730=CARTESIAN_POINT ( 'NONE',  ( 12.49999999999993960, 2.500000000000000000, 4.330127018922196314 ) ) ;
#122731=FACE_OUTER_BOUND ( 'NONE', #60498, .T. ) ;
#122732=ORIENTED_EDGE ( 'NONE', *, *, #102954, .T. ) ;
#122733=ORIENTED_EDGE ( 'NONE', *, *, #52414, .T. ) ;
#122734=DIRECTION ( 'NONE',  ( 0.000000000000000000, 0.000000000000000000, -1.000000000000000000 ) ) ;
#122735=FACE_OUTER_BOUND ( 'NONE', #20090, .T. ) ;
#122736=CARTESIAN_POINT ( 'NONE',  ( 0.1999999999999627909, 12.50000000000000000, 0.3464101615137758494 ) ) ;
#122737=FACE_OUTER_BOUND ( 'NONE', #66443, .T. ) ;
#122738=CARTESIAN_POINT ( 'NONE',  ( 14.34999999999989306, 12.50000000000000000, -1.818653347947326138 ) ) ;
#122739=CONICAL_SURFACE ( 'NONE', #118527, 0.1000000000000002554, 0.003490658503988666988 ) ;
#122740=ORIENTED_EDGE ( 'NONE', *, *, #18555, .F. ) ;
#122741=EDGE_CURVE ( 'NONE', #65687, #127955, #89511, .T. ) ;
#122742=DIRECTION ( 'NONE',  ( 0.000000000000000000, 0.000000000000000000, 1.000000000000000000 ) ) ;
#122743=ORIENTED_EDGE ( 'NONE', *, *, #93943, .F. ) ;
#122744=DIRECTION ( 'NONE',  ( 0.000000000000000000, 1.000000000000000000, 0.000000000000000000 ) ) ;
#122745=EDGE_CURVE ( 'NONE', #119361, #14309, #102134, .T. ) ;
#122746=ORIENTED_EDGE ( 'NONE', *, *, #73044, .T. ) ;
#122747=LINE ( 'NONE', #22633, #92296 ) ;
#122748=LINE ( 'NONE', #73005, #44856 ) ;
#122750=CARTESIAN_POINT ( 'NONE',  ( -2.100000000000033396, 2.500000000000000000, -3.637306695894650055 ) ) ;
#122751=EDGE_CURVE ( 'NONE', #15438, #50878, #118848, .T. ) ;
#122752=PLANE ( 'NONE',  #108628 ) ;
#122753=EDGE_LOOP ( 'NONE', ( #82777, #123159, #122050, #41832 ) ) ;
#122754=EDGE_CURVE ( 'NONE', #27176, #82484, #91662, .T. ) ;
#122755=LINE ( 'NONE', #110351, #96931 ) ;
#122756=CIRCLE ( 'NONE', #112298, 0.09999999999999982514 ) ;
#122757=AXIS2_PLACEMENT_3D ( 'NONE', #78206, #28462, #38947 ) ;
#122758=EDGE_CURVE ( 'NONE', #9515, #118519, #112506, .T. ) ;
#122759=DIRECTION ( 'NONE',  ( 0.000000000000000000, 0.000000000000000000, 1.000000000000000000 ) ) ;
#122760=ORIENTED_EDGE ( 'NONE', *, *, #7323, .T. ) ;
#122761=ORIENTED_EDGE ( 'NONE', *, *, #98551, .T. ) ;
#122762=ORIENTED_EDGE ( 'NONE', *, *, #59486, .T. ) ;
#122763=FACE_OUTER_BOUND ( 'NONE', #48956, .T. ) ;
#122766=DIRECTION ( 'NONE',  ( 0.000000000000000000, 0.000000000000000000, 1.000000000000000000 ) ) ;
#122767=EDGE_CURVE ( 'NONE', #45205, #76614, #33104, .T. ) ;
#122769=DIRECTION ( 'NONE',  ( 0.000000000000000000, 1.000000000000000000, 0.000000000000000000 ) ) ;
#122770=AXIS2_PLACEMENT_3D ( 'NONE', #128270, #98781, #9121 ) ;
#122771=CONICAL_SURFACE ( 'NONE', #39265, 0.1000000000000002554, 0.003490658503988666988 ) ;
#122772=DIRECTION ( 'NONE',  ( 0.000000000000000000, -0.000000000000000000, 1.000000000000000000 ) ) ;
#122773=CARTESIAN_POINT ( 'NONE',  ( -12.69999999999999396, 12.50000000000000000, -4.048810130592460865 ) ) ;
#122774=CONICAL_SURFACE ( 'NONE', #9903, 0.1000000000000002554, 0.003490658503988666988 ) ;
#122775=DIRECTION ( 'NONE',  ( 0.000000000000000000, 0.000000000000000000, -1.000000000000000000 ) ) ;
#122776=VECTOR ( 'NONE', #42710, 1000.000000000000000 ) ;
#122777=ORIENTED_EDGE ( 'NONE', *, *, #19538, .T. ) ;
#122778=CARTESIAN_POINT ( 'NONE',  ( -4.250072516143177381E-14, 12.50000000000000000, -3.637306695894650055 ) ) ;
#122779=DIRECTION ( 'NONE',  ( -0.000000000000000000, -1.000000000000000000, -0.000000000000000000 ) ) ;
#122780=EDGE_CURVE ( 'NONE', #10245, #39901, #24407, .T. ) ;
#122781=DIRECTION ( 'NONE',  ( 0.000000000000000000, -0.000000000000000000, 1.000000000000000000 ) ) ;
#122782=CARTESIAN_POINT ( 'NONE',  ( 2.949999999999945111, 2.500000000000000000, 2.265063509461097357 ) ) ;
#122783=EDGE_LOOP ( 'NONE', ( #5278, #54181, #3468, #89181 ) ) ;
#122784=DIRECTION ( 'NONE',  ( -0.000000000000000000, 1.000000000000000000, -0.000000000000000000 ) ) ;
#122785=CIRCLE ( 'NONE', #110258, 0.1000000000000002554 ) ;
#122786=LINE ( 'NONE', #13462, #65958 ) ;
#122787=CARTESIAN_POINT ( 'NONE',  ( 2.099999999999950351, 2.500000000000000000, -2.276824562219559311E-15 ) ) ;
#122788=EDGE_LOOP ( 'NONE', ( #29925, #66901 ) ) ;
#122789=AXIS2_PLACEMENT_3D ( 'NONE', #112262, #44152, #91321 ) ;
#122790=AXIS2_PLACEMENT_3D ( 'NONE', #117050, #9703, #27383 ) ;
#122791=VERTEX_POINT ( 'NONE', #64330 ) ;
#122792=CONICAL_SURFACE ( 'NONE', #89347, 0.1000000000000002554, 0.003490658503988666988 ) ;
#122793=DIRECTION ( 'NONE',  ( 0.000000000000000000, 0.000000000000000000, -1.000000000000000000 ) ) ;
#122794=CIRCLE ( 'NONE', #68406, 0.06509327318403745899 ) ;
#122795=EDGE_CURVE ( 'NONE', #98740, #68909, #45700, .T. ) ;
#122796=ORIENTED_EDGE ( 'NONE', *, *, #46458, .F. ) ;
#122797=ORIENTED_EDGE ( 'NONE', *, *, #65633, .T. ) ;
#122798=DIRECTION ( 'NONE',  ( -0.000000000000000000, 1.000000000000000000, -0.000000000000000000 ) ) ;
#122799=AXIS2_PLACEMENT_3D ( 'NONE', #116729, #15295, #27079 ) ;
#122800=ORIENTED_EDGE ( 'NONE', *, *, #44800, .T. ) ;
#122801=CARTESIAN_POINT ( 'NONE',  ( -5.200000000000024158, 2.500000000000000000, -4.676537180435977881 ) ) ;
#122802=DIRECTION ( 'NONE',  ( -4.274815082592931898E-19, -0.9999939076577903929, -0.003490651415223739937 ) ) ;
#122803=AXIS2_PLACEMENT_3D ( 'NONE', #24655, #95966, #116241 ) ;
#122804=CARTESIAN_POINT ( 'NONE',  ( -6.050000000000020250, 2.500000000000000000, -6.841600689897078702 ) ) ;
#122805=VERTEX_POINT ( 'NONE', #123255 ) ;
#122806=AXIS2_PLACEMENT_3D ( 'NONE', #83792, #76557, #13749 ) ;
#122807=AXIS2_PLACEMENT_3D ( 'NONE', #1891, #49731, #19608 ) ;
#122808=DIRECTION ( 'NONE',  ( -0.000000000000000000, -1.000000000000000000, -0.000000000000000000 ) ) ;
#122810=VERTEX_POINT ( 'NONE', #86542 ) ;
#122811=CARTESIAN_POINT ( 'NONE',  ( 17.41715230668771852, 1.872943439152341183, 4.643388583733590202 ) ) ;
#122812=AXIS2_PLACEMENT_3D ( 'NONE', #109183, #10354, #19524 ) ;
#122813=EDGE_CURVE ( 'NONE', #58229, #70966, #31048, .T. ) ;
#122814=DIRECTION ( 'NONE',  ( 0.000000000000000000, 0.000000000000000000, -1.000000000000000000 ) ) ;
#122815=ORIENTED_EDGE ( 'NONE', *, *, #26963, .F. ) ;
#122816=AXIS2_PLACEMENT_3D ( 'NONE', #65080, #95216, #5517 ) ;
#122817=AXIS2_PLACEMENT_3D ( 'NONE', #101297, #86461, #47202 ) ;
#122818=ORIENTED_EDGE ( 'NONE', *, *, #98480, .F. ) ;
#122819=EDGE_LOOP ( 'NONE', ( #110568, #127573, #107119, #80250 ) ) ;
#122820=VERTEX_POINT ( 'NONE', #46616 ) ;
#122821=DIRECTION ( 'NONE',  ( -0.000000000000000000, -1.000000000000000000, -0.000000000000000000 ) ) ;
#122822=CARTESIAN_POINT ( 'NONE',  ( 13.51931942373995099, 2.499999999999999112, 8.074217332245385848 ) ) ;
#122824=DIRECTION ( 'NONE',  ( 0.000000000000000000, 0.000000000000000000, 1.000000000000000000 ) ) ;
#122825=FACE_BOUND ( 'NONE', #62956, .T. ) ;
#122826=ORIENTED_EDGE ( 'NONE', *, *, #54173, .T. ) ;
#122828=DIRECTION ( 'NONE',  ( -0.000000000000000000, 1.000000000000000000, -0.000000000000000000 ) ) ;
#122829=DIRECTION ( 'NONE',  ( 0.000000000000000000, 1.000000000000000000, 0.000000000000000000 ) ) ;
#122830=CARTESIAN_POINT ( 'NONE',  ( -6.450000000000019718, 2.500000000000000000, -1.818653347947326138 ) ) ;
#122831=FACE_OUTER_BOUND ( 'NONE', #24940, .T. ) ;
#122832=AXIS2_PLACEMENT_3D ( 'NONE', #35292, #115096, #25432 ) ;
#122833=CARTESIAN_POINT ( 'NONE',  ( 3.749999999999975131, 2.500000000000000000, 6.495190528383297135 ) ) ;
#122834=CARTESIAN_POINT ( 'NONE',  ( -8.550000000000011369, 2.500000000000000000, 1.918653347947321564 ) ) ;
#122835=ADVANCED_FACE ( 'NONE', ( #7329 ), #64464, .T. ) ;
#122836=EDGE_LOOP ( 'NONE', ( #10360, #19745 ) ) ;
#122838=EDGE_LOOP ( 'NONE', ( #55130, #104216, #61344, #67733 ) ) ;
#122839=ORIENTED_EDGE ( 'NONE', *, *, #117260, .T. ) ;
#122840=EDGE_LOOP ( 'NONE', ( #7370, #66085, #62206, #76956 ) ) ;
#122841=CARTESIAN_POINT ( 'NONE',  ( 12.29999999999990656, 12.50000000000000000, -4.676537180435977881 ) ) ;
#122842=DIRECTION ( 'NONE',  ( 0.000000000000000000, 1.000000000000000000, 0.000000000000000000 ) ) ;
#122843=VERTEX_POINT ( 'NONE', #108114 ) ;
#122844=FACE_BOUND ( 'NONE', #74982, .T. ) ;
#122845=CARTESIAN_POINT ( 'NONE',  ( 7.299999999999924327, 2.500000000000000000, 0.2464101615137735679 ) ) ;
#122846=EDGE_CURVE ( 'NONE', #119087, #76531, #116644, .T. ) ;
#122847=VECTOR ( 'NONE', #2146, 1000.000000000000000 ) ;
#122848=VECTOR ( 'NONE', #121990, 1000.000000000000000 ) ;
#122849=ORIENTED_EDGE ( 'NONE', *, *, #47067, .T. ) ;
#122850=EDGE_CURVE ( 'NONE', #55169, #77714, #89125, .T. ) ;
#122851=FACE_OUTER_BOUND ( 'NONE', #113246, .T. ) ;
#122852=EDGE_CURVE ( 'NONE', #1184, #30745, #26994, .T. ) ;
#122853=DIRECTION ( 'NONE',  ( 0.000000000000000000, 1.000000000000000000, 0.000000000000000000 ) ) ;
#122854=EDGE_CURVE ( 'NONE', #92073, #126313, #16326, .T. ) ;
#122855=FACE_OUTER_BOUND ( 'NONE', #109514, .T. ) ;
#122856=EDGE_CURVE ( 'NONE', #1725, #95822, #97009, .T. ) ;
#122857=ORIENTED_EDGE ( 'NONE', *, *, #37875, .F. ) ;
#122858=LINE ( 'NONE', #92092, #57613 ) ;
#122859=EDGE_LOOP ( 'NONE', ( #38308, #79878 ) ) ;
#122860=AXIS2_PLACEMENT_3D ( 'NONE', #67481, #117226, #47241 ) ;
#122861=CONICAL_SURFACE ( 'NONE', #49720, 0.1000000000000002554, 0.003490658503988666988 ) ;
#122862=EDGE_CURVE ( 'NONE', #112423, #84654, #58230, .T. ) ;
#122863=ORIENTED_EDGE ( 'NONE', *, *, #71564, .T. ) ;
#122864=EDGE_CURVE ( 'NONE', #32927, #23200, #106238, .T. ) ;
#122865=VERTEX_POINT ( 'NONE', #37463 ) ;
#122866=DIRECTION ( 'NONE',  ( 0.000000000000000000, 1.000000000000000000, 0.000000000000000000 ) ) ;
#122868=CARTESIAN_POINT ( 'NONE',  ( -5.650000000000019895, 12.50000000000000000, 2.511473670974873507 ) ) ;
#122869=ORIENTED_EDGE ( 'NONE', *, *, #75856, .F. ) ;
#122870=EDGE_CURVE ( 'NONE', #35208, #49210, #107479, .T. ) ;
#122871=DIRECTION ( 'NONE',  ( 0.000000000000000000, -0.9999939076577903929, 0.003490651415223739937 ) ) ;
#122872=ADVANCED_FACE ( 'NONE', ( #126481 ), #99987, .T. ) ;
#122873=AXIS2_PLACEMENT_3D ( 'NONE', #100780, #39956, #111239 ) ;
#122874=FACE_OUTER_BOUND ( 'NONE', #20223, .T. ) ;
#122875=EDGE_CURVE ( 'NONE', #48799, #37790, #27605, .T. ) ;
#122876=CARTESIAN_POINT ( 'NONE',  ( -12.49999999999999289, 2.500000000000000000, 5.022947341949748790 ) ) ;
#122879=CARTESIAN_POINT ( 'NONE',  ( 2.299999999999946976, 2.500000000000000000, 4.776537180435972196 ) ) ;
#122880=EDGE_CURVE ( 'NONE', #124753, #76648, #78012, .T. ) ;
#122881=ORIENTED_EDGE ( 'NONE', *, *, #58416, .F. ) ;
#122882=DIRECTION ( 'NONE',  ( 0.000000000000000000, -0.000000000000000000, 1.000000000000000000 ) ) ;
#122883=CONICAL_SURFACE ( 'NONE', #93633, 0.09999999999999982514, 0.003490658503988666988 ) ;
#122884=ORIENTED_EDGE ( 'NONE', *, *, #10416, .T. ) ;
#122885=ORIENTED_EDGE ( 'NONE', *, *, #78087, .F. ) ;
#122886=CARTESIAN_POINT ( 'NONE',  ( 11.64999999999990798, 2.500000000000000000, 5.902370205355745192 ) ) ;
#122887=AXIS2_PLACEMENT_3D ( 'NONE', #79251, #117857, #88392 ) ;
#122888=DIRECTION ( 'NONE',  ( -0.000000000000000000, 1.000000000000000000, -0.000000000000000000 ) ) ;
#122889=CARTESIAN_POINT ( 'NONE',  ( -5.400000000000020783, 12.50000000000000000, 0.6928203230275494784 ) ) ;
#122890=DIRECTION ( 'NONE',  ( 0.000000000000000000, 0.000000000000000000, -1.000000000000000000 ) ) ;
#122891=DIRECTION ( 'NONE',  ( 0.000000000000000000, 1.000000000000000000, 0.000000000000000000 ) ) ;
#122892=CIRCLE ( 'NONE', #81129, 0.1000000000000000472 ) ;
#122893=EDGE_LOOP ( 'NONE', ( #126158, #54444 ) ) ;
#122894=VECTOR ( 'NONE', #115131, 1000.000000000000000 ) ;
#122895=ORIENTED_EDGE ( 'NONE', *, *, #108983, .T. ) ;
#122896=PLANE ( 'NONE',  #64220 ) ;
#122897=AXIS2_PLACEMENT_3D ( 'NONE', #102361, #12661, #63069 ) ;
#122898=DIRECTION ( 'NONE',  ( 0.000000000000000000, 1.000000000000000000, 0.000000000000000000 ) ) ;
#122899=FACE_OUTER_BOUND ( 'NONE', #38115, .T. ) ;
#122900=ORIENTED_EDGE ( 'NONE', *, *, #54126, .T. ) ;
#122901=ORIENTED_EDGE ( 'NONE', *, *, #91088, .F. ) ;
#122902=DIRECTION ( 'NONE',  ( 0.000000000000000000, -0.000000000000000000, 1.000000000000000000 ) ) ;
#122903=CONICAL_SURFACE ( 'NONE', #9932, 0.1000000000000002554, 0.003490658503988666988 ) ;
#122904=ORIENTED_EDGE ( 'NONE', *, *, #48870, .F. ) ;
#122905=PLANE ( 'NONE',  #65417 ) ;
#122906=CARTESIAN_POINT ( 'NONE',  ( -10.40000000000000213, 2.500000000000000000, -4.330127018922197202 ) ) ;
#122907=CIRCLE ( 'NONE', #14121, 0.1000000000000002554 ) ;
#122908=CARTESIAN_POINT ( 'NONE',  ( 1.849999999999949685, 12.50000000000000000, 1.818653347947321475 ) ) ;
#122909=ORIENTED_EDGE ( 'NONE', *, *, #41928, .F. ) ;
#122910=DIRECTION ( 'NONE',  ( 0.000000000000000000, -0.9999939076577903929, 0.003490651415223739937 ) ) ;
#122911=CARTESIAN_POINT ( 'NONE',  ( 12.49999999999993605, 2.500000000000000000, -2.276824562219559311E-15 ) ) ;
#122912=CARTESIAN_POINT ( 'NONE',  ( 9.149999999999918643, 12.50000000000000000, -6.495190528383302464 ) ) ;
#122913=FACE_OUTER_BOUND ( 'NONE', #87108, .T. ) ;
#122914=AXIS2_PLACEMENT_3D ( 'NONE', #117546, #48192, #37095 ) ;
#122915=DIRECTION ( 'NONE',  ( 0.000000000000000000, -0.000000000000000000, 1.000000000000000000 ) ) ;
#122916=ORIENTED_EDGE ( 'NONE', *, *, #49537, .T. ) ;
#122917=ADVANCED_FACE ( 'NONE', ( #18451 ), #98288, .T. ) ;
#122918=DIRECTION ( 'NONE',  ( 0.000000000000000000, 0.000000000000000000, -1.000000000000000000 ) ) ;
#122919=AXIS2_PLACEMENT_3D ( 'NONE', #2805, #20526, #101664 ) ;
#122920=AXIS2_PLACEMENT_3D ( 'NONE', #86799, #25284, #125440 ) ;
#122921=DIRECTION ( 'NONE',  ( 0.000000000000000000, 1.000000000000000000, 0.000000000000000000 ) ) ;
#122922=EDGE_CURVE ( 'NONE', #20150, #88083, #52057, .T. ) ;
#122923=ORIENTED_EDGE ( 'NONE', *, *, #36547, .F. ) ;
#122924=ORIENTED_EDGE ( 'NONE', *, *, #108437, .F. ) ;
#122926=CARTESIAN_POINT ( 'NONE',  ( 14.34999999999989306, 2.500000000000000000, -1.718653347947326049 ) ) ;
#122927=CARTESIAN_POINT ( 'NONE',  ( -1.700000000000035261, 2.500000000000000000, 4.230127018922196669 ) ) ;
#122928=DIRECTION ( 'NONE',  ( -0.000000000000000000, -1.000000000000000000, -0.000000000000000000 ) ) ;
#122929=EDGE_CURVE ( 'NONE', #81018, #123846, #118573, .T. ) ;
#122930=DIRECTION ( 'NONE',  ( 0.000000000000000000, 0.000000000000000000, 1.000000000000000000 ) ) ;
#122931=DIRECTION ( 'NONE',  ( 0.000000000000000000, 1.000000000000000000, 0.000000000000000000 ) ) ;
#122932=DIRECTION ( 'NONE',  ( 0.000000000000000000, 0.000000000000000000, 1.000000000000000000 ) ) ;
#122933=CARTESIAN_POINT ( 'NONE',  ( 11.24999999999990585, 12.50000000000000000, 2.857883832488649301 ) ) ;
#122934=LINE ( 'NONE', #65276, #108387 ) ;
#122935=DIRECTION ( 'NONE',  ( 0.000000000000000000, -0.000000000000000000, 1.000000000000000000 ) ) ;
#122936=EDGE_LOOP ( 'NONE', ( #41279, #15648, #35324, #116603 ) ) ;
#122937=EDGE_LOOP ( 'NONE', ( #29707, #26194, #44754, #67743 ) ) ;
#122938=VERTEX_POINT ( 'NONE', #59024 ) ;
#122939=CONICAL_SURFACE ( 'NONE', #12186, 0.1000000000000000472, 0.003490658503988666988 ) ;
#122940=CONICAL_SURFACE ( 'NONE', #3801, 0.1000000000000002554, 0.003490658503988666988 ) ;
#122941=ORIENTED_EDGE ( 'NONE', *, *, #122387, .F. ) ;
#122942=CARTESIAN_POINT ( 'NONE',  ( 11.64999999999990443, 12.50000000000000000, 2.857883832488649301 ) ) ;
#122943=DIRECTION ( 'NONE',  ( 0.000000000000000000, 0.000000000000000000, -1.000000000000000000 ) ) ;
#122944=EDGE_LOOP ( 'NONE', ( #74606, #107182, #55501, #77227 ) ) ;
#122945=VECTOR ( 'NONE', #25646, 1000.000000000000000 ) ;
#122946=CARTESIAN_POINT ( 'NONE',  ( 4.349999999999938360, 2.500000000000000000, 1.818653347947321475 ) ) ;
#122947=CIRCLE ( 'NONE', #37180, 0.06509327318403745899 ) ;
#122948=DIRECTION ( 'NONE',  ( -4.274815082592931898E-19, -0.9999939076577903929, -0.003490651415223739937 ) ) ;
#122950=ORIENTED_EDGE ( 'NONE', *, *, #79295, .T. ) ;
#122951=DIRECTION ( 'NONE',  ( 0.000000000000000000, 0.000000000000000000, 1.000000000000000000 ) ) ;
#122952=CIRCLE ( 'NONE', #49806, 0.06509327318403745899 ) ;
#122953=DIRECTION ( 'NONE',  ( 0.000000000000000000, -0.9999939076577903929, 0.003490651415223739937 ) ) ;
#122954=ORIENTED_EDGE ( 'NONE', *, *, #4770, .F. ) ;
#122955=AXIS2_PLACEMENT_3D ( 'NONE', #111989, #3315, #123094 ) ;
#122956=ORIENTED_EDGE ( 'NONE', *, *, #36254, .T. ) ;
#122957=ORIENTED_EDGE ( 'NONE', *, *, #45197, .F. ) ;
#122958=EDGE_LOOP ( 'NONE', ( #1947, #124777, #99474, #74850 ) ) ;
#122959=FACE_OUTER_BOUND ( 'NONE', #119444, .T. ) ;
#122960=DIRECTION ( 'NONE',  ( 0.000000000000000000, 0.000000000000000000, -1.000000000000000000 ) ) ;
#122961=CARTESIAN_POINT ( 'NONE',  ( 13.94999999999989626, 12.50000000000000000, 2.576566944158910744 ) ) ;
#122962=DIRECTION ( 'NONE',  ( -0.000000000000000000, -1.000000000000000000, -0.000000000000000000 ) ) ;
#122963=AXIS2_PLACEMENT_3D ( 'NONE', #56198, #76502, #77141 ) ;
#122964=VERTEX_POINT ( 'NONE', #98946 ) ;
#122965=CARTESIAN_POINT ( 'NONE',  ( -2.900000000000030109, 12.50000000000000000, -3.572213422710612374 ) ) ;
#122966=ADVANCED_FACE ( 'NONE', ( #9279 ), #45797, .T. ) ;
#122967=VERTEX_POINT ( 'NONE', #69471 ) ;
#122968=VECTOR ( 'NONE', #77377, 1000.000000000000000 ) ;
#122969=LINE ( 'NONE', #23470, #85197 ) ;
#122970=DIRECTION ( 'NONE',  ( -0.000000000000000000, 1.000000000000000000, -0.000000000000000000 ) ) ;
#122971=FACE_OUTER_BOUND ( 'NONE', #78458, .T. ) ;
#122972=DIRECTION ( 'NONE',  ( 0.000000000000000000, 0.000000000000000000, 1.000000000000000000 ) ) ;
#122973=EDGE_CURVE ( 'NONE', #29920, #28513, #43652, .T. ) ;
#122974=ORIENTED_EDGE ( 'NONE', *, *, #13986, .T. ) ;
#122975=CIRCLE ( 'NONE', #33109, 0.06509327318403745899 ) ;
#122976=VECTOR ( 'NONE', #38216, 1000.000000000000000 ) ;
#122977=ORIENTED_EDGE ( 'NONE', *, *, #101753, .F. ) ;
#122978=VERTEX_POINT ( 'NONE', #10545 ) ;
#122979=CARTESIAN_POINT ( 'NONE',  ( -3.150000000000029665, 2.500000000000000000, 6.841600689897072485 ) ) ;
#122980=CARTESIAN_POINT ( 'NONE',  ( -5.850000000000019185, 2.500000000000000000, 2.065063509461097624 ) ) ;
#122981=EDGE_CURVE ( 'NONE', #28898, #105571, #100073, .T. ) ;
#122982=DIRECTION ( 'NONE',  ( 0.000000000000000000, 1.000000000000000000, 0.000000000000000000 ) ) ;
#122983=FACE_BOUND ( 'NONE', #35693, .T. ) ;
#122984=CARTESIAN_POINT ( 'NONE',  ( 10.84999999999991260, 12.50000000000000000, 5.802370205355744659 ) ) ;
#122985=DIRECTION ( 'NONE',  ( 0.000000000000000000, 0.000000000000000000, 1.000000000000000000 ) ) ;
#122986=AXIS2_PLACEMENT_3D ( 'NONE', #17594, #21980, #80890 ) ;
#122987=CARTESIAN_POINT ( 'NONE',  ( -12.69999999999999396, 2.500000000000000000, 0.4464101615137776591 ) ) ;
#122988=CONICAL_SURFACE ( 'NONE', #77008, 0.1000000000000002554, 0.003490658503988666988 ) ;
#122990=DIRECTION ( 'NONE',  ( -0.000000000000000000, -1.000000000000000000, -0.000000000000000000 ) ) ;
#122991=AXIS2_PLACEMENT_3D ( 'NONE', #127056, #114638, #46538 ) ;
#122992=LINE ( 'NONE', #113160, #9293 ) ;
#122993=ORIENTED_EDGE ( 'NONE', *, *, #127512, .T. ) ;
#122994=DIRECTION ( 'NONE',  ( 0.000000000000000000, 0.000000000000000000, -1.000000000000000000 ) ) ;
#122995=ADVANCED_FACE ( 'NONE', ( #32157 ), #101527, .T. ) ;
#122996=VERTEX_POINT ( 'NONE', #111997 ) ;
#122997=VERTEX_POINT ( 'NONE', #81246 ) ;
#122998=VECTOR ( 'NONE', #66642, 1000.000000000000000 ) ;
#123000=FACE_BOUND ( 'NONE', #12302, .T. ) ;
#123001=CARTESIAN_POINT ( 'NONE',  ( -4.550000000000026468, 2.500000000000000000, -6.495190528383302464 ) ) ;
#123002=ADVANCED_FACE ( 'NONE', ( #121161 ), #95954, .T. ) ;
#123003=AXIS2_PLACEMENT_3D ( 'NONE', #63348, #122921, #92820 ) ;
#123004=AXIS2_PLACEMENT_3D ( 'NONE', #33472, #113297, #11870 ) ;
#123005=ORIENTED_EDGE ( 'NONE', *, *, #75693, .F. ) ;
#123006=EDGE_CURVE ( 'NONE', #114427, #56742, #64555, .T. ) ;
#123007=CARTESIAN_POINT ( 'NONE',  ( 59.88087687670552128, 3.776023963378999149, 4.996435080099743686 ) ) ;
#123008=EDGE_CURVE ( 'NONE', #50768, #29262, #125203, .T. ) ;
#123009=LINE ( 'NONE', #73257, #93859 ) ;
#123010=EDGE_CURVE ( 'NONE', #28226, #108826, #8121, .T. ) ;
#123011=EDGE_CURVE ( 'NONE', #104378, #118365, #84294, .T. ) ;
#123012=EDGE_LOOP ( 'NONE', ( #16290, #46159 ) ) ;
#123013=LINE ( 'NONE', #33362, #46933 ) ;
#123014=FACE_OUTER_BOUND ( 'NONE', #65151, .T. ) ;
#123015=EDGE_CURVE ( 'NONE', #7925, #4623, #26907, .T. ) ;
#123016=EDGE_LOOP ( 'NONE', ( #49418, #51063 ) ) ;
#123017=VECTOR ( 'NONE', #93543, 1000.000000000000000 ) ;
#123019=EDGE_CURVE ( 'NONE', #76567, #72606, #41604, .T. ) ;
#123020=DIRECTION ( 'NONE',  ( 0.000000000000000000, -0.000000000000000000, 1.000000000000000000 ) ) ;
#123021=EDGE_LOOP ( 'NONE', ( #19613, #104034 ) ) ;
#123022=AXIS2_PLACEMENT_3D ( 'NONE', #80611, #118579, #68842 ) ;
#123023=DIRECTION ( 'NONE',  ( 0.000000000000000000, 0.000000000000000000, -1.000000000000000000 ) ) ;
#123024=ADVANCED_FACE ( 'NONE', ( #30870 ), #94117, .T. ) ;
#123025=VECTOR ( 'NONE', #64151, 1000.000000000000000 ) ;
#123026=DIRECTION ( 'NONE',  ( -0.000000000000000000, -1.000000000000000000, -0.000000000000000000 ) ) ;
#123027=CIRCLE ( 'NONE', #47818, 0.06509327318403741736 ) ;
#123028=DIRECTION ( 'NONE',  ( 0.000000000000000000, -0.000000000000000000, 1.000000000000000000 ) ) ;
#123029=ORIENTED_EDGE ( 'NONE', *, *, #57991, .T. ) ;
#123030=VERTEX_POINT ( 'NONE', #11194 ) ;
#123031=EDGE_CURVE ( 'NONE', #113064, #56167, #112603, .T. ) ;
#123032=DIRECTION ( 'NONE',  ( 0.000000000000000000, 1.000000000000000000, 0.000000000000000000 ) ) ;
#123033=EDGE_CURVE ( 'NONE', #27106, #129486, #70141, .T. ) ;
#123034=VECTOR ( 'NONE', #8874, 1000.000000000000000 ) ;
#123035=VERTEX_POINT ( 'NONE', #60946 ) ;
#123036=CARTESIAN_POINT ( 'NONE',  ( -5.400000000000020783, 12.50000000000000000, 5.022947341949748790 ) ) ;
#123037=LINE ( 'NONE', #43848, #20139 ) ;
#123038=CONICAL_SURFACE ( 'NONE', #62410, 0.1000000000000002554, 0.003490658503988666988 ) ;
#123039=EDGE_LOOP ( 'NONE', ( #11277, #51707, #104503, #24964 ) ) ;
#123040=CARTESIAN_POINT ( 'NONE',  ( -0.6500000000000398792, 12.50000000000000000, -2.511473670974877948 ) ) ;
#123041=DIRECTION ( 'NONE',  ( 0.000000000000000000, 0.000000000000000000, -1.000000000000000000 ) ) ;
#123043=DIRECTION ( 'NONE',  ( 0.000000000000000000, -0.9999939076577903929, 0.003490651415223739937 ) ) ;
#123044=CARTESIAN_POINT ( 'NONE',  ( -11.64999999999999680, 2.500000000000000000, 6.495190528383297135 ) ) ;
#123045=ORIENTED_EDGE ( 'NONE', *, *, #34383, .F. ) ;
#123046=CONICAL_SURFACE ( 'NONE', #120989, 0.1000000000000002554, 0.003490658503988666988 ) ;
#123047=VERTEX_POINT ( 'NONE', #1375 ) ;
#123048=LINE ( 'NONE', #72020, #13948 ) ;
#123049=VERTEX_POINT ( 'NONE', #51149 ) ;
#123050=DIRECTION ( 'NONE',  ( 0.000000000000000000, 1.000000000000000000, 0.000000000000000000 ) ) ;
#123051=ORIENTED_EDGE ( 'NONE', *, *, #326, .F. ) ;
#123052=ORIENTED_EDGE ( 'NONE', *, *, #55869, .F. ) ;
#123053=ORIENTED_EDGE ( 'NONE', *, *, #124067, .F. ) ;
#123054=DIRECTION ( 'NONE',  ( -0.000000000000000000, -1.000000000000000000, -0.000000000000000000 ) ) ;
#123055=CIRCLE ( 'NONE', #108461, 0.06509327318403745899 ) ;
#123056=DIRECTION ( 'NONE',  ( 0.000000000000000000, 1.000000000000000000, 0.000000000000000000 ) ) ;
#123057=DIRECTION ( 'NONE',  ( 0.000000000000000000, -0.000000000000000000, 1.000000000000000000 ) ) ;
#123058=DIRECTION ( 'NONE',  ( 0.000000000000000000, 0.000000000000000000, 1.000000000000000000 ) ) ;
#123059=LINE ( 'NONE', #13076, #48173 ) ;
#123060=CIRCLE ( 'NONE', #62430, 0.06509327318403745899 ) ;
#123062=DIRECTION ( 'NONE',  ( 0.000000000000000000, 1.000000000000000000, 0.000000000000000000 ) ) ;
#123063=AXIS2_PLACEMENT_3D ( 'NONE', #45031, #47604, #104577 ) ;
#123064=DIRECTION ( 'NONE',  ( 0.000000000000000000, 0.000000000000000000, 1.000000000000000000 ) ) ;
#123065=DIRECTION ( 'NONE',  ( 0.000000000000000000, 1.000000000000000000, 0.000000000000000000 ) ) ;
#123066=EDGE_LOOP ( 'NONE', ( #38259, #122640, #105812, #3425 ) ) ;
#123067=ADVANCED_FACE ( 'NONE', ( #54200 ), #110530, .T. ) ;
#123069=EDGE_CURVE ( 'NONE', #16889, #19644, #33192, .T. ) ;
#123070=CARTESIAN_POINT ( 'NONE',  ( 9.999999999999948486, 2.500000000000000000, -4.430127018922202176 ) ) ;
#123071=EDGE_LOOP ( 'NONE', ( #89836, #793 ) ) ;
#123072=ORIENTED_EDGE ( 'NONE', *, *, #70132, .F. ) ;
#123073=DIRECTION ( 'NONE',  ( 0.000000000000000000, 0.000000000000000000, 1.000000000000000000 ) ) ;
#123074=DIRECTION ( 'NONE',  ( -0.000000000000000000, 1.000000000000000000, -0.000000000000000000 ) ) ;
#123075=CIRCLE ( 'NONE', #26926, 0.1000000000000002554 ) ;
#123076=DIRECTION ( 'NONE',  ( -0.000000000000000000, 1.000000000000000000, -0.000000000000000000 ) ) ;
#123077=DIRECTION ( 'NONE',  ( 0.000000000000000000, 1.000000000000000000, 0.000000000000000000 ) ) ;
#123078=CIRCLE ( 'NONE', #47869, 0.09999999999999999167 ) ;
#123079=DIRECTION ( 'NONE',  ( -0.000000000000000000, 1.000000000000000000, -0.000000000000000000 ) ) ;
#123080=DIRECTION ( 'NONE',  ( -0.000000000000000000, 1.000000000000000000, -0.000000000000000000 ) ) ;
#123081=CARTESIAN_POINT ( 'NONE',  ( -3.550000000000028244, 2.500000000000000000, 2.511473670974873507 ) ) ;
#123082=VERTEX_POINT ( 'NONE', #121795 ) ;
#123083=DIRECTION ( 'NONE',  ( 0.000000000000000000, -0.9999939076577903929, 0.003490651415223739937 ) ) ;
#123084=AXIS2_PLACEMENT_3D ( 'NONE', #103075, #13395, #104991 ) ;
#123085=DIRECTION ( 'NONE',  ( 0.000000000000000000, 0.000000000000000000, -1.000000000000000000 ) ) ;
#123086=ORIENTED_EDGE ( 'NONE', *, *, #55037, .F. ) ;
#123087=ORIENTED_EDGE ( 'NONE', *, *, #35679, .T. ) ;
#123088=AXIS2_PLACEMENT_3D ( 'NONE', #40700, #70774, #60948 ) ;
#123089=AXIS2_PLACEMENT_3D ( 'NONE', #62144, #119751, #70654 ) ;
#123090=VERTEX_POINT ( 'NONE', #34575 ) ;
#123091=VECTOR ( 'NONE', #113020, 1000.000000000000000 ) ;
#123092=ORIENTED_EDGE ( 'NONE', *, *, #10518, .F. ) ;
#123094=DIRECTION ( 'NONE',  ( 0.000000000000000000, -0.000000000000000000, 1.000000000000000000 ) ) ;
#123095=VECTOR ( 'NONE', #33039, 1000.000000000000000 ) ;
#123096=AXIS2_PLACEMENT_3D ( 'NONE', #75147, #82412, #122330 ) ;
#123097=CARTESIAN_POINT ( 'NONE',  ( 4.199999999999941558, 2.500000000000000000, -4.330127018922201643 ) ) ;
#123098=CARTESIAN_POINT ( 'NONE',  ( 7.299999999999926104, 12.50000000000000000, -3.918623584224389056 ) ) ;
#123099=DIRECTION ( 'NONE',  ( 0.000000000000000000, 1.000000000000000000, 0.000000000000000000 ) ) ;
#123100=ORIENTED_EDGE ( 'NONE', *, *, #58048, .T. ) ;
#123101=DIRECTION ( 'NONE',  ( 0.000000000000000000, 0.000000000000000000, 1.000000000000000000 ) ) ;
#123102=CARTESIAN_POINT ( 'NONE',  ( -12.69999999999999218, 12.50000000000000000, -4.611443907251937091 ) ) ;
#123103=FACE_OUTER_BOUND ( 'NONE', #18800, .T. ) ;
#123104=DIRECTION ( 'NONE',  ( 0.000000000000000000, 0.000000000000000000, -1.000000000000000000 ) ) ;
#123105=EDGE_CURVE ( 'NONE', #119556, #87886, #74481, .T. ) ;
#123106=ORIENTED_EDGE ( 'NONE', *, *, #124039, .T. ) ;
#123107=ORIENTED_EDGE ( 'NONE', *, *, #64731, .T. ) ;
#123108=ORIENTED_EDGE ( 'NONE', *, *, #5771, .F. ) ;
#123109=AXIS2_PLACEMENT_3D ( 'NONE', #105940, #77128, #16243 ) ;
#123110=CARTESIAN_POINT ( 'NONE',  ( -6.650000000000018119, 2.500000000000000000, -6.395190528383301931 ) ) ;
#123111=DIRECTION ( 'NONE',  ( -4.274815082592931898E-19, -0.9999939076577903929, -0.003490651415223739937 ) ) ;
#123112=DIRECTION ( 'NONE',  ( -0.000000000000000000, -1.000000000000000000, -0.000000000000000000 ) ) ;
#123113=EDGE_CURVE ( 'NONE', #22205, #110118, #114729, .T. ) ;
#123114=CONICAL_SURFACE ( 'NONE', #74993, 0.09999999999999982514, 0.003490658503988666988 ) ;
#123115=CIRCLE ( 'NONE', #66658, 0.1000000000000002554 ) ;
#123116=ADVANCED_FACE ( 'NONE', ( #84937 ), #54099, .T. ) ;
#123117=ORIENTED_EDGE ( 'NONE', *, *, #40558, .F. ) ;
#123118=DIRECTION ( 'NONE',  ( 0.000000000000000000, 0.000000000000000000, -1.000000000000000000 ) ) ;
#123119=CARTESIAN_POINT ( 'NONE',  ( -7.500000000000016875, 2.500000000000000000, -3.537306695894649966 ) ) ;
#123120=CARTESIAN_POINT ( 'NONE',  ( 5.799999999999934985, 2.500000000000000000, -4.330127018922201643 ) ) ;
#123121=ADVANCED_FACE ( 'NONE', ( #65934 ), #35215, .T. ) ;
#123122=CARTESIAN_POINT ( 'NONE',  ( -11.05000000000000071, 2.500000000000000000, 6.741600689897071952 ) ) ;
#123123=AXIS2_PLACEMENT_3D ( 'NONE', #10083, #50034, #80767 ) ;
#123124=CIRCLE ( 'NONE', #24829, 0.06509327318403745899 ) ;
#123125=AXIS2_PLACEMENT_3D ( 'NONE', #85545, #75716, #70424 ) ;
#123126=DIRECTION ( 'NONE',  ( -0.000000000000000000, -1.000000000000000000, -0.000000000000000000 ) ) ;
#123127=EDGE_LOOP ( 'NONE', ( #31225, #93798 ) ) ;
#123128=EDGE_LOOP ( 'NONE', ( #124015, #86149 ) ) ;
#123129=EDGE_CURVE ( 'NONE', #113061, #86174, #62528, .T. ) ;
#123130=CARTESIAN_POINT ( 'NONE',  ( -1.050000000000038236, 2.500000000000000000, -6.048780366869526581 ) ) ;
#123131=DIRECTION ( 'NONE',  ( -0.000000000000000000, 1.000000000000000000, -0.000000000000000000 ) ) ;
#123132=CIRCLE ( 'NONE', #79330, 0.06509327318403745899 ) ;
#123133=CARTESIAN_POINT ( 'NONE',  ( 21.23528140090977345, 2.699413673072321718, -2.293764360948945757 ) ) ;
#123134=DIRECTION ( 'NONE',  ( -4.274815082592931898E-19, -0.9999939076577903929, -0.003490651415223739937 ) ) ;
#123135=CARTESIAN_POINT ( 'NONE',  ( 10.19999999999991580, 2.500000000000000000, -0.4464101615137783252 ) ) ;
#123136=VECTOR ( 'NONE', #23440, 1000.000000000000000 ) ;
#123137=ORIENTED_EDGE ( 'NONE', *, *, #105591, .F. ) ;
#123138=ORIENTED_EDGE ( 'NONE', *, *, #70827, .T. ) ;
#123139=DIRECTION ( 'NONE',  ( -0.000000000000000000, 1.000000000000000000, -0.000000000000000000 ) ) ;
#123140=DIRECTION ( 'NONE',  ( 0.000000000000000000, -0.000000000000000000, 1.000000000000000000 ) ) ;
#123141=DIRECTION ( 'NONE',  ( 0.000000000000000000, 1.000000000000000000, 0.000000000000000000 ) ) ;
#123142=DIRECTION ( 'NONE',  ( -0.000000000000000000, 1.000000000000000000, -0.000000000000000000 ) ) ;
#123143=CARTESIAN_POINT ( 'NONE',  ( -12.69999999999999218, 2.500000000000000000, 4.576537180435972019 ) ) ;
#123144=EDGE_LOOP ( 'NONE', ( #17871, #79158, #85008, #9260 ) ) ;
#123145=AXIS2_PLACEMENT_3D ( 'NONE', #30329, #61049, #70880 ) ;
#123146=DIRECTION ( 'NONE',  ( 0.000000000000000000, 0.000000000000000000, -1.000000000000000000 ) ) ;
#123147=CARTESIAN_POINT ( 'NONE',  ( -9.350000000000004974, 2.500000000000000000, 6.741600689897071952 ) ) ;
#123148=AXIS2_PLACEMENT_3D ( 'NONE', #40368, #67867, #18770 ) ;
#123149=ORIENTED_EDGE ( 'NONE', *, *, #119429, .T. ) ;
#123150=DIRECTION ( 'NONE',  ( 0.000000000000000000, 1.000000000000000000, 0.000000000000000000 ) ) ;
#123151=ORIENTED_EDGE ( 'NONE', *, *, #32015, .F. ) ;
#123152=DIRECTION ( 'NONE',  ( -0.000000000000000000, -1.000000000000000000, -0.000000000000000000 ) ) ;
#123153=EDGE_CURVE ( 'NONE', #4134, #33730, #124872, .T. ) ;
#123154=ORIENTED_EDGE ( 'NONE', *, *, #83833, .T. ) ;
#123155=AXIS2_PLACEMENT_3D ( 'NONE', #3629, #31812, #112304 ) ;
#123156=DIRECTION ( 'NONE',  ( 0.000000000000000000, 0.000000000000000000, 1.000000000000000000 ) ) ;
#123157=DIRECTION ( 'NONE',  ( 0.000000000000000000, 0.000000000000000000, -1.000000000000000000 ) ) ;
#123158=ORIENTED_EDGE ( 'NONE', *, *, #40337, .F. ) ;
#123159=ORIENTED_EDGE ( 'NONE', *, *, #23139, .T. ) ;
#123160=EDGE_CURVE ( 'NONE', #9507, #37294, #16811, .T. ) ;
#123162=CARTESIAN_POINT ( 'NONE',  ( -4.800000000000022915, 12.50000000000000000, -0.3464101615137783474 ) ) ;
#123163=VECTOR ( 'NONE', #26965, 1000.000000000000000 ) ;
#123164=EDGE_CURVE ( 'NONE', #89915, #58166, #76417, .T. ) ;
#123167=CIRCLE ( 'NONE', #129458, 0.1000000000000002554 ) ;
#123168=DIRECTION ( 'NONE',  ( 0.000000000000000000, -0.000000000000000000, 1.000000000000000000 ) ) ;
#123169=CARTESIAN_POINT ( 'NONE',  ( 8.149999999999920419, 2.500000000000000000, 6.148780366869520897 ) ) ;
#123170=EDGE_CURVE ( 'NONE', #64066, #378, #127273, .T. ) ;
#123171=EDGE_CURVE ( 'NONE', #119497, #54885, #22819, .T. ) ;
#123172=DIRECTION ( 'NONE',  ( -0.000000000000000000, 1.000000000000000000, -0.000000000000000000 ) ) ;
#123173=CARTESIAN_POINT ( 'NONE',  ( -11.44999999999999751, 2.500000000000000000, 2.511473670974873507 ) ) ;
#123174=CIRCLE ( 'NONE', #35351, 0.1000000000000000472 ) ;
#123175=EDGE_CURVE ( 'NONE', #79817, #20424, #66609, .T. ) ;
#123176=ADVANCED_FACE ( 'NONE', ( #46293 ), #47849, .T. ) ;
#123177=ORIENTED_EDGE ( 'NONE', *, *, #54434, .F. ) ;
#123178=EDGE_LOOP ( 'NONE', ( #44747, #59065 ) ) ;
#123179=DIRECTION ( 'NONE',  ( 0.000000000000000000, 1.000000000000000000, 0.000000000000000000 ) ) ;
#123180=CIRCLE ( 'NONE', #20770, 0.1000000000000002554 ) ;
#123181=ADVANCED_FACE ( 'NONE', ( #106511 ), #104273, .T. ) ;
#123183=CARTESIAN_POINT ( 'NONE',  ( 1.849999999999949019, 2.500000000000000000, 6.841600689897072485 ) ) ;
#123184=PLANE ( 'NONE',  #1052 ) ;
#123185=DIRECTION ( 'NONE',  ( 0.000000000000000000, 0.000000000000000000, -1.000000000000000000 ) ) ;
#123186=AXIS2_PLACEMENT_3D ( 'NONE', #74237, #2928, #62501 ) ;
#123187=ORIENTED_EDGE ( 'NONE', *, *, #60253, .F. ) ;
#123189=FACE_BOUND ( 'NONE', #82560, .T. ) ;
#123190=ORIENTED_EDGE ( 'NONE', *, *, #29087, .T. ) ;
#123191=CARTESIAN_POINT ( 'NONE',  ( -9.400000000000009237, 2.500000000000000000, -3.883716857408422207 ) ) ;
#123192=DIRECTION ( 'NONE',  ( -0.000000000000000000, 1.000000000000000000, -0.000000000000000000 ) ) ;
#123193=EDGE_CURVE ( 'NONE', #70406, #104107, #25355, .T. ) ;
#123194=CARTESIAN_POINT ( 'NONE',  ( -10.20000000000000462, 2.500000000000000000, 0.2464101615137735679 ) ) ;
#123195=AXIS2_PLACEMENT_3D ( 'NONE', #45658, #23414, #25342 ) ;
#123197=CARTESIAN_POINT ( 'NONE',  ( 4.399999999999937295, 2.500000000000000000, 4.676537180435972552 ) ) ;
#123198=LINE ( 'NONE', #36100, #20068 ) ;
#123199=DIRECTION ( 'NONE',  ( -0.000000000000000000, -1.000000000000000000, -0.000000000000000000 ) ) ;
#123200=CARTESIAN_POINT ( 'NONE',  ( 12.09999999999990550, 2.500000000000000000, -4.330127018922201643 ) ) ;
#123201=CARTESIAN_POINT ( 'NONE',  ( 8.349999999999923261, 2.500000000000000000, 2.957883832488649389 ) ) ;
#123202=DIRECTION ( 'NONE',  ( -0.000000000000000000, 1.000000000000000000, -0.000000000000000000 ) ) ;
#123203=DIRECTION ( 'NONE',  ( 0.000000000000000000, -0.9999939076577903929, 0.003490651415223739937 ) ) ;
#123204=CARTESIAN_POINT ( 'NONE',  ( -11.89999999999999503, 2.500000000000000000, 4.576537180435972019 ) ) ;
#123205=ORIENTED_EDGE ( 'NONE', *, *, #128917, .T. ) ;
#123206=VERTEX_POINT ( 'NONE', #77056 ) ;
#123207=ORIENTED_EDGE ( 'NONE', *, *, #72228, .F. ) ;
#123208=LINE ( 'NONE', #69745, #111740 ) ;
#123209=ORIENTED_EDGE ( 'NONE', *, *, #31221, .F. ) ;
#123210=DIRECTION ( 'NONE',  ( -0.000000000000000000, -1.000000000000000000, -0.000000000000000000 ) ) ;
#123211=ORIENTED_EDGE ( 'NONE', *, *, #47704, .T. ) ;
#123212=ORIENTED_EDGE ( 'NONE', *, *, #84455, .F. ) ;
#123213=ORIENTED_EDGE ( 'NONE', *, *, #124232, .F. ) ;
#123215=CIRCLE ( 'NONE', #89751, 0.1000000000000002554 ) ;
#123216=CONICAL_SURFACE ( 'NONE', #110587, 0.1000000000000002554, 0.003490658503988666988 ) ;
#123217=DIRECTION ( 'NONE',  ( 0.000000000000000000, -0.000000000000000000, 1.000000000000000000 ) ) ;
#123218=CARTESIAN_POINT ( 'NONE',  ( -7.050000000000016698, 2.500000000000000000, -2.165063509461101710 ) ) ;
#123219=CARTESIAN_POINT ( 'NONE',  ( -6.450000000000019718, 12.50000000000000000, -1.818653347947326138 ) ) ;
#123220=CARTESIAN_POINT ( 'NONE',  ( 1.649999999999951505, 2.500000000000000000, -2.857883832488653741 ) ) ;
#123221=ORIENTED_EDGE ( 'NONE', *, *, #124276, .F. ) ;
#123222=AXIS2_PLACEMENT_3D ( 'NONE', #6667, #116650, #25054 ) ;
#123223=CIRCLE ( 'NONE', #127424, 0.06509327318403745899 ) ;
#123224=CARTESIAN_POINT ( 'NONE',  ( -10.40000000000000213, 2.500000000000000000, 4.230127018922196669 ) ) ;
#123225=ORIENTED_EDGE ( 'NONE', *, *, #36165, .T. ) ;
#123226=AXIS2_PLACEMENT_3D ( 'NONE', #73293, #113878, #123667 ) ;
#123227=EDGE_LOOP ( 'NONE', ( #28698, #126253 ) ) ;
#123228=EDGE_CURVE ( 'NONE', #3365, #82926, #1857, .T. ) ;
#123229=VERTEX_POINT ( 'NONE', #96046 ) ;
#123230=DIRECTION ( 'NONE',  ( 0.000000000000000000, 0.000000000000000000, 1.000000000000000000 ) ) ;
#123231=ORIENTED_EDGE ( 'NONE', *, *, #67265, .T. ) ;
#123232=ORIENTED_EDGE ( 'NONE', *, *, #14793, .T. ) ;
#123233=VERTEX_POINT ( 'NONE', #87498 ) ;
#123235=CIRCLE ( 'NONE', #129517, 0.1000000000000002554 ) ;
#123236=DIRECTION ( 'NONE',  ( 0.000000000000000000, 1.000000000000000000, 0.000000000000000000 ) ) ;
#123237=PLANE ( 'NONE',  #45893 ) ;
#123238=CIRCLE ( 'NONE', #77257, 0.06509327318403745899 ) ;
#123239=DIRECTION ( 'NONE',  ( 0.000000000000000000, -0.9999939076577903929, 0.003490651415223739937 ) ) ;
#123240=DIRECTION ( 'NONE',  ( -0.000000000000000000, 1.000000000000000000, -0.000000000000000000 ) ) ;
#123241=DIRECTION ( 'NONE',  ( 0.000000000000000000, 0.000000000000000000, 1.000000000000000000 ) ) ;
#123242=LINE ( 'NONE', #35510, #44757 ) ;
#123243=ORIENTED_EDGE ( 'NONE', *, *, #7436, .T. ) ;
#123244=CARTESIAN_POINT ( 'NONE',  ( 15.83209681635555022, 2.500000000000000000, -5.404881881984143099 ) ) ;
#123245=VERTEX_POINT ( 'NONE', #67192 ) ;
#123247=AXIS2_PLACEMENT_3D ( 'NONE', #24303, #45237, #53758 ) ;
#123248=ORIENTED_EDGE ( 'NONE', *, *, #70676, .F. ) ;
#123249=ORIENTED_EDGE ( 'NONE', *, *, #101847, .F. ) ;
#123250=DIRECTION ( 'NONE',  ( -4.274815082592931898E-19, -0.9999939076577903929, -0.003490651415223739937 ) ) ;
#123251=DIRECTION ( 'NONE',  ( -0.000000000000000000, -1.000000000000000000, -0.000000000000000000 ) ) ;
#123252=DIRECTION ( 'NONE',  ( -0.000000000000000000, 1.000000000000000000, -0.000000000000000000 ) ) ;
#123253=VERTEX_POINT ( 'NONE', #15538 ) ;
#123254=ORIENTED_EDGE ( 'NONE', *, *, #108417, .T. ) ;
#123255=CARTESIAN_POINT ( 'NONE',  ( -15.59999999999998010, 12.50000000000000000, 0.4115034346978133639 ) ) ;
#123256=CARTESIAN_POINT ( 'NONE',  ( -11.84999999999999787, 12.50000000000000000, -1.753560074763284460 ) ) ;
#123257=CARTESIAN_POINT ( 'NONE',  ( 12.89999999999990266, 2.500000000000000000, 5.122947341949749323 ) ) ;
#123258=CARTESIAN_POINT ( 'NONE',  ( 13.09999999999990195, 2.500000000000000000, 4.083716857408420609 ) ) ;
#123259=DIRECTION ( 'NONE',  ( 0.000000000000000000, -0.9999939076577903929, 0.003490651415223739937 ) ) ;
#123260=EDGE_CURVE ( 'NONE', #26010, #81531, #33285, .T. ) ;
#123261=ORIENTED_EDGE ( 'NONE', *, *, #126420, .T. ) ;
#123262=AXIS2_PLACEMENT_3D ( 'NONE', #59147, #96459, #118691 ) ;
#123263=VERTEX_POINT ( 'NONE', #35844 ) ;
#123264=CARTESIAN_POINT ( 'NONE',  ( 6.449999999999931788, 12.50000000000000000, 6.148780366869520009 ) ) ;
#123265=DIRECTION ( 'NONE',  ( 0.000000000000000000, -0.000000000000000000, 1.000000000000000000 ) ) ;
#123266=ADVANCED_FACE ( 'NONE', ( #115679 ), #16177, .T. ) ;
#123267=AXIS2_PLACEMENT_3D ( 'NONE', #82869, #95262, #52742 ) ;
#123268=CIRCLE ( 'NONE', #62737, 0.1000000000000000472 ) ;
#123269=CIRCLE ( 'NONE', #33410, 0.06509327318403745899 ) ;
#123270=ADVANCED_FACE ( 'NONE', ( #6347 ), #75120, .T. ) ;
#123272=CARTESIAN_POINT ( 'NONE',  ( 8.749999999999923617, 2.500000000000000000, -7.288010851410854585 ) ) ;
#123273=CARTESIAN_POINT ( 'NONE',  ( 4.149999999999941735, 12.50000000000000000, -2.857883832488653741 ) ) ;
#123274=DIRECTION ( 'NONE',  ( -4.274815082592931898E-19, -0.9999939076577903929, -0.003490651415223739937 ) ) ;
#123275=EDGE_CURVE ( 'NONE', #105827, #16102, #87629, .T. ) ;
#123276=DIRECTION ( 'NONE',  ( -0.000000000000000000, 1.000000000000000000, -0.000000000000000000 ) ) ;
#123277=VERTEX_POINT ( 'NONE', #88127 ) ;
#123278=CIRCLE ( 'NONE', #27137, 0.06509327318403745899 ) ;
#123279=DIRECTION ( 'NONE',  ( 0.000000000000000000, 0.000000000000000000, -1.000000000000000000 ) ) ;
#123280=DIRECTION ( 'NONE',  ( -0.000000000000000000, -1.000000000000000000, -0.000000000000000000 ) ) ;
#123281=DIRECTION ( 'NONE',  ( -0.000000000000000000, 1.000000000000000000, -0.000000000000000000 ) ) ;
#123282=ADVANCED_FACE ( 'NONE', ( #90077 ), #58070, .T. ) ;
#123283=EDGE_LOOP ( 'NONE', ( #66157, #22508, #6266, #40591 ) ) ;
#123284=EDGE_CURVE ( 'NONE', #88991, #74504, #48238, .T. ) ;
#123285=FACE_OUTER_BOUND ( 'NONE', #22998, .T. ) ;
#123286=ORIENTED_EDGE ( 'NONE', *, *, #45608, .T. ) ;
#123287=CARTESIAN_POINT ( 'NONE',  ( 2.699999999999944666, 12.50000000000000000, 4.676537180435972552 ) ) ;
#123288=ORIENTED_EDGE ( 'NONE', *, *, #125777, .T. ) ;
#123289=LINE ( 'NONE', #64992, #58499 ) ;
#123290=FACE_OUTER_BOUND ( 'NONE', #82227, .T. ) ;
#123291=DIRECTION ( 'NONE',  ( -0.000000000000000000, -1.000000000000000000, -0.000000000000000000 ) ) ;
#123292=ORIENTED_EDGE ( 'NONE', *, *, #89888, .F. ) ;
#123293=CIRCLE ( 'NONE', #45946, 0.06509327318403745899 ) ;
#123294=DIRECTION ( 'NONE',  ( -0.000000000000000000, -1.000000000000000000, -0.000000000000000000 ) ) ;
#123296=CARTESIAN_POINT ( 'NONE',  ( 3.549999999999942091, 12.50000000000000000, 2.446380397790835826 ) ) ;
#123297=EDGE_LOOP ( 'NONE', ( #60545, #22343, #6278, #81444 ) ) ;
#123298=AXIS2_PLACEMENT_3D ( 'NONE', #103762, #14705, #63839 ) ;
#123299=AXIS2_PLACEMENT_3D ( 'NONE', #12597, #83916, #63657 ) ;
#123300=EDGE_LOOP ( 'NONE', ( #102930, #54532 ) ) ;
#123301=ORIENTED_EDGE ( 'NONE', *, *, #76024, .T. ) ;
#123302=CARTESIAN_POINT ( 'NONE',  ( 1.249999999999953815, 2.500000000000000000, 1.472243186433545459 ) ) ;
#123303=DIRECTION ( 'NONE',  ( 0.000000000000000000, -0.9999939076577903929, 0.003490651415223739937 ) ) ;
#123304=DIRECTION ( 'NONE',  ( -4.274815082592931898E-19, -0.9999939076577903929, -0.003490651415223739937 ) ) ;
#123305=VERTEX_POINT ( 'NONE', #19405 ) ;
#123306=CIRCLE ( 'NONE', #66868, 0.06509327318403745899 ) ;
#123307=DIRECTION ( 'NONE',  ( 0.000000000000000000, 0.000000000000000000, 1.000000000000000000 ) ) ;
#123308=CARTESIAN_POINT ( 'NONE',  ( -7.500000000000015099, 2.500000000000000000, -5.022947341949754119 ) ) ;
#123309=EDGE_LOOP ( 'NONE', ( #104623, #79545 ) ) ;
#123310=AXIS2_PLACEMENT_3D ( 'NONE', #36830, #96361, #115350 ) ;
#123311=CARTESIAN_POINT ( 'NONE',  ( -3.550000000000027356, 2.500000000000000000, -2.511473670974877948 ) ) ;
#123312=CARTESIAN_POINT ( 'NONE',  ( 9.149999999999918643, 2.500000000000000000, -6.495190528383302464 ) ) ;
#123313=AXIS2_PLACEMENT_3D ( 'NONE', #33481, #125690, #25559 ) ;
#123314=DIRECTION ( 'NONE',  ( 0.000000000000000000, 1.000000000000000000, 0.000000000000000000 ) ) ;
#123315=ADVANCED_FACE ( 'NONE', ( #97975 ), #50014, .T. ) ;
#123316=PLANE ( 'NONE',  #28353 ) ;
#123317=CARTESIAN_POINT ( 'NONE',  ( -0.8500000000000382805, 12.50000000000000000, -5.802370205355749988 ) ) ;
#123318=EDGE_CURVE ( 'NONE', #53598, #82164, #31220, .T. ) ;
#123319=AXIS2_PLACEMENT_3D ( 'NONE', #127067, #68121, #108053 ) ;
#123320=DIRECTION ( 'NONE',  ( 0.000000000000000000, 1.000000000000000000, 0.000000000000000000 ) ) ;
#123321=CARTESIAN_POINT ( 'NONE',  ( 2.299999999999947864, 12.50000000000000000, 3.983716857408420964 ) ) ;
#123322=EDGE_CURVE ( 'NONE', #62381, #17095, #68512, .T. ) ;
#123323=AXIS2_PLACEMENT_3D ( 'NONE', #5271, #57617, #105423 ) ;
#123324=EDGE_CURVE ( 'NONE', #98051, #113165, #102320, .T. ) ;
#123325=EDGE_LOOP ( 'NONE', ( #125031, #19448, #17166, #54297 ) ) ;
#123326=ORIENTED_EDGE ( 'NONE', *, *, #113985, .T. ) ;
#123327=EDGE_CURVE ( 'NONE', #117845, #100514, #108435, .T. ) ;
#123328=VERTEX_POINT ( 'NONE', #39735 ) ;
#123329=ORIENTED_EDGE ( 'NONE', *, *, #66979, .F. ) ;
#123330=AXIS2_PLACEMENT_3D ( 'NONE', #98831, #9174, #49116 ) ;
#123331=LINE ( 'NONE', #33664, #16048 ) ;
#123332=DIRECTION ( 'NONE',  ( -0.000000000000000000, 1.000000000000000000, -0.000000000000000000 ) ) ;
#123333=LINE ( 'NONE', #100467, #82306 ) ;
#123334=VERTEX_POINT ( 'NONE', #118908 ) ;
#123335=FACE_BOUND ( 'NONE', #105941, .T. ) ;
#123336=DIRECTION ( 'NONE',  ( 0.000000000000000000, -0.000000000000000000, 1.000000000000000000 ) ) ;
#123337=DIRECTION ( 'NONE',  ( 0.000000000000000000, 0.000000000000000000, -1.000000000000000000 ) ) ;
#123338=ADVANCED_FACE ( 'NONE', ( #20074 ), #9600, .T. ) ;
#123339=FACE_OUTER_BOUND ( 'NONE', #78518, .T. ) ;
#123340=EDGE_CURVE ( 'NONE', #54140, #87803, #117590, .T. ) ;
#123341=DIRECTION ( 'NONE',  ( -4.274815082592931898E-19, -0.9999939076577903929, -0.003490651415223739937 ) ) ;
#123342=DIRECTION ( 'NONE',  ( -0.000000000000000000, 1.000000000000000000, -0.000000000000000000 ) ) ;
#123343=FACE_OUTER_BOUND ( 'NONE', #40284, .T. ) ;
#123344=DIRECTION ( 'NONE',  ( 0.000000000000000000, 0.000000000000000000, -1.000000000000000000 ) ) ;
#123345=CARTESIAN_POINT ( 'NONE',  ( -4.250072516143177381E-14, 12.50000000000000000, -3.572213422710612374 ) ) ;
#123347=CARTESIAN_POINT ( 'NONE',  ( 4.549999999999939426, 2.500000000000000000, -2.065063509461102065 ) ) ;
#123348=ORIENTED_EDGE ( 'NONE', *, *, #66837, .T. ) ;
#123349=EDGE_LOOP ( 'NONE', ( #68739, #127047 ) ) ;
#123350=ORIENTED_EDGE ( 'NONE', *, *, #108524, .T. ) ;
#123351=ORIENTED_EDGE ( 'NONE', *, *, #81346, .T. ) ;
#123352=ORIENTED_EDGE ( 'NONE', *, *, #45304, .T. ) ;
#123353=EDGE_LOOP ( 'NONE', ( #114822, #90166 ) ) ;
#123354=DIRECTION ( 'NONE',  ( -0.000000000000000000, 1.000000000000000000, -0.000000000000000000 ) ) ;
#123355=CONICAL_SURFACE ( 'NONE', #98206, 0.09999999999999982514, 0.003490658503988666988 ) ;
#123356=VERTEX_POINT ( 'NONE', #89450 ) ;
#123357=VERTEX_POINT ( 'NONE', #129408 ) ;
#123358=CONICAL_SURFACE ( 'NONE', #10473, 0.1000000000000002554, 0.003490658503988666988 ) ;
#123359=AXIS2_PLACEMENT_3D ( 'NONE', #50088, #99816, #81464 ) ;
#123360=CARTESIAN_POINT ( 'NONE',  ( 15.62882261213625235, -2.499999999999999556, 5.624357572923363691 ) ) ;
#123361=DIRECTION ( 'NONE',  ( -0.000000000000000000, 1.000000000000000000, -0.000000000000000000 ) ) ;
#123362=CARTESIAN_POINT ( 'NONE',  ( 9.799999999999917222, 2.500000000000000000, 0.3464101615137735735 ) ) ;
#123363=VERTEX_POINT ( 'NONE', #39087 ) ;
#123364=LINE ( 'NONE', #36776, #81945 ) ;
#123365=AXIS2_PLACEMENT_3D ( 'NONE', #76731, #66255, #116647 ) ;
#123366=ORIENTED_EDGE ( 'NONE', *, *, #124509, .F. ) ;
#123367=ORIENTED_EDGE ( 'NONE', *, *, #53575, .F. ) ;
#123368=DIRECTION ( 'NONE',  ( -0.000000000000000000, -1.000000000000000000, -0.000000000000000000 ) ) ;
#123369=DIRECTION ( 'NONE',  ( 0.000000000000000000, 0.000000000000000000, 1.000000000000000000 ) ) ;
#123370=ORIENTED_EDGE ( 'NONE', *, *, #6445, .F. ) ;
#123371=ORIENTED_EDGE ( 'NONE', *, *, #76044, .T. ) ;
#123372=CARTESIAN_POINT ( 'NONE',  ( -10.00000000000000533, 12.50000000000000000, -5.022947341949749678 ) ) ;
#123373=ADVANCED_FACE ( 'NONE', ( #79008 ), #52140, .T. ) ;
#123374=CARTESIAN_POINT ( 'NONE',  ( -1.250000000000035749, 12.50000000000000000, -2.857883832488653741 ) ) ;
#123375=PLANE ( 'NONE',  #74958 ) ;
#123376=DIRECTION ( 'NONE',  ( 0.000000000000000000, 0.000000000000000000, 1.000000000000000000 ) ) ;
#123378=VERTEX_POINT ( 'NONE', #18121 ) ;
#123379=CARTESIAN_POINT ( 'NONE',  ( 2.500000000000002220, -2.500000000000000000, 9.000000000000001776 ) ) ;
#123380=CIRCLE ( 'NONE', #66929, 0.06509327318403743123 ) ;
#123381=CIRCLE ( 'NONE', #6287, 0.06509327318403745899 ) ;
#123382=ORIENTED_EDGE ( 'NONE', *, *, #51328, .T. ) ;
#123383=CARTESIAN_POINT ( 'NONE',  ( 11.84999999999990727, 2.500000000000000000, 6.048780366869520364 ) ) ;
#123384=ORIENTED_EDGE ( 'NONE', *, *, #73588, .F. ) ;
#123385=CARTESIAN_POINT ( 'NONE',  ( 8.349999999999919709, 2.500000000000000000, 5.802370205355744659 ) ) ;
#123386=DIRECTION ( 'NONE',  ( -4.274815082592931898E-19, -0.9999939076577903929, -0.003490651415223739937 ) ) ;
#123388=DIRECTION ( 'NONE',  ( 0.000000000000000000, 0.000000000000000000, 1.000000000000000000 ) ) ;
#123389=VERTEX_POINT ( 'NONE', #69815 ) ;
#123390=CONICAL_SURFACE ( 'NONE', #33528, 0.09999999999999982514, 0.003490658503988666988 ) ;
#123391=DIRECTION ( 'NONE',  ( -4.274815082592931898E-19, -0.9999939076577903929, -0.003490651415223739937 ) ) ;
#123392=EDGE_LOOP ( 'NONE', ( #122646, #54157, #37811, #117233 ) ) ;
#123393=ORIENTED_EDGE ( 'NONE', *, *, #10807, .T. ) ;
#123394=EDGE_LOOP ( 'NONE', ( #19975, #24485, #26428, #39629 ) ) ;
#123395=CARTESIAN_POINT ( 'NONE',  ( 17.50000000000000000, 2.749999999999999556, 10.00000000000000178 ) ) ;
#123396=DIRECTION ( 'NONE',  ( 0.000000000000000000, 1.000000000000000000, 0.000000000000000000 ) ) ;
#123398=DIRECTION ( 'NONE',  ( 0.000000000000000000, 0.000000000000000000, 1.000000000000000000 ) ) ;
#123399=AXIS2_PLACEMENT_3D ( 'NONE', #13785, #123112, #102188 ) ;
#123400=AXIS2_PLACEMENT_3D ( 'NONE', #64691, #45072, #45711 ) ;
#123401=DIRECTION ( 'NONE',  ( -0.000000000000000000, -1.000000000000000000, -0.000000000000000000 ) ) ;
#123402=CARTESIAN_POINT ( 'NONE',  ( -1.900000000000034550, 12.50000000000000000, 4.676537180435972552 ) ) ;
#123403=EDGE_CURVE ( 'NONE', #28777, #128265, #114818, .T. ) ;
#123404=AXIS2_PLACEMENT_3D ( 'NONE', #39917, #60835, #59576 ) ;
#123405=ORIENTED_EDGE ( 'NONE', *, *, #10814, .T. ) ;
#123406=FACE_OUTER_BOUND ( 'NONE', #34022, .T. ) ;
#123407=ADVANCED_FACE ( 'NONE', ( #50192 ), #116867, .T. ) ;
#123408=ORIENTED_EDGE ( 'NONE', *, *, #69497, .F. ) ;
#123409=AXIS2_PLACEMENT_3D ( 'NONE', #126705, #65831, #126039 ) ;
#123410=DIRECTION ( 'NONE',  ( 0.000000000000000000, 0.000000000000000000, 1.000000000000000000 ) ) ;
#123411=EDGE_CURVE ( 'NONE', #98982, #86533, #37569, .T. ) ;
#123412=DIRECTION ( 'NONE',  ( 0.000000000000000000, -0.000000000000000000, 1.000000000000000000 ) ) ;
#123413=DIRECTION ( 'NONE',  ( -0.000000000000000000, 1.000000000000000000, -0.000000000000000000 ) ) ;
#123414=DIRECTION ( 'NONE',  ( 0.000000000000000000, -0.9999939076577903929, 0.003490651415223739937 ) ) ;
#123415=EDGE_CURVE ( 'NONE', #46680, #102274, #77180, .T. ) ;
#123416=VERTEX_POINT ( 'NONE', #104988 ) ;
#123417=DIRECTION ( 'NONE',  ( 0.000000000000000000, 0.000000000000000000, 1.000000000000000000 ) ) ;
#123418=DIRECTION ( 'NONE',  ( 0.000000000000000000, 0.000000000000000000, -1.000000000000000000 ) ) ;
#123419=ORIENTED_EDGE ( 'NONE', *, *, #106183, .T. ) ;
#123420=EDGE_CURVE ( 'NONE', #108043, #43147, #79340, .T. ) ;
#123421=EDGE_CURVE ( 'NONE', #6735, #76595, #127863, .T. ) ;
#123422=EDGE_CURVE ( 'NONE', #86459, #40320, #129436, .T. ) ;
#123423=ADVANCED_FACE ( 'NONE', ( #96455 ), #24943, .T. ) ;
#123424=EDGE_CURVE ( 'NONE', #86712, #67418, #72977, .T. ) ;
#123425=ORIENTED_EDGE ( 'NONE', *, *, #110161, .F. ) ;
#123426=CARTESIAN_POINT ( 'NONE',  ( 10.19999999999991225, 12.50000000000000000, -4.741630453620016006 ) ) ;
#123427=EDGE_LOOP ( 'NONE', ( #108342, #107173, #48846, #73889 ) ) ;
#123428=EDGE_LOOP ( 'NONE', ( #41258, #74305 ) ) ;
#123429=CARTESIAN_POINT ( 'NONE',  ( 97.50000000000000000, 0.000000000000000000, 0.000000000000000000 ) ) ;
#123430=AXIS2_PLACEMENT_3D ( 'NONE', #71064, #110964, #12126 ) ;
#123431=AXIS2_PLACEMENT_3D ( 'NONE', #111789, #60752, #51587 ) ;
#123432=ADVANCED_FACE ( 'NONE', ( #15314 ), #7438, .T. ) ;
#123433=ORIENTED_EDGE ( 'NONE', *, *, #113546, .T. ) ;
#123434=CARTESIAN_POINT ( 'NONE',  ( 16.84158739990415654, 0.4722467112503249131, -5.802037699230074175 ) ) ;
#123435=CARTESIAN_POINT ( 'NONE',  ( 1.049999999999953637, 12.50000000000000000, -1.818653347947326138 ) ) ;
#123436=DIRECTION ( 'NONE',  ( 0.000000000000000000, 0.000000000000000000, 1.000000000000000000 ) ) ;
#123437=ORIENTED_EDGE ( 'NONE', *, *, #117831, .F. ) ;
#123438=AXIS2_PLACEMENT_3D ( 'NONE', #94441, #95106, #4762 ) ;
#123439=DIRECTION ( 'NONE',  ( 0.000000000000000000, -0.9999939076577903929, 0.003490651415223739937 ) ) ;
#123440=DIRECTION ( 'NONE',  ( 0.000000000000000000, 1.000000000000000000, 0.000000000000000000 ) ) ;
#123441=VERTEX_POINT ( 'NONE', #118040 ) ;
#123442=LINE ( 'NONE', #114905, #50688 ) ;
#123443=DIRECTION ( 'NONE',  ( 0.000000000000000000, -0.9999939076577903929, 0.003490651415223739937 ) ) ;
#123444=VERTEX_POINT ( 'NONE', #76198 ) ;
#123445=ORIENTED_EDGE ( 'NONE', *, *, #122447, .T. ) ;
#123446=EDGE_LOOP ( 'NONE', ( #36950, #83543 ) ) ;
#123447=VERTEX_POINT ( 'NONE', #6146 ) ;
#123448=CARTESIAN_POINT ( 'NONE',  ( 11.04999999999990656, 2.500000000000000000, -6.148780366869526226 ) ) ;
#123449=DIRECTION ( 'NONE',  ( 0.000000000000000000, 0.000000000000000000, 1.000000000000000000 ) ) ;
#123450=CARTESIAN_POINT ( 'NONE',  ( 3.949999999999940670, 2.500000000000000000, 1.818653347947321475 ) ) ;
#123451=FACE_BOUND ( 'NONE', #26955, .T. ) ;
#123452=EDGE_LOOP ( 'NONE', ( #117505, #66781, #48542, #125368 ) ) ;
#123454=CARTESIAN_POINT ( 'NONE',  ( 6.899999999999928413, 12.50000000000000000, 3.983716857408420964 ) ) ;
#123455=DIRECTION ( 'NONE',  ( 0.000000000000000000, 0.000000000000000000, -1.000000000000000000 ) ) ;
#123456=DIRECTION ( 'NONE',  ( 0.000000000000000000, 0.000000000000000000, 1.000000000000000000 ) ) ;
#123457=CARTESIAN_POINT ( 'NONE',  ( 2.499999999999947153, 12.50000000000000000, 0.6277270498435120194 ) ) ;
#123458=EDGE_CURVE ( 'NONE', #56145, #128265, #95190, .T. ) ;
#123459=DIRECTION ( 'NONE',  ( -4.274815082592931898E-19, -0.9999939076577903929, -0.003490651415223739937 ) ) ;
#123460=EDGE_CURVE ( 'NONE', #76430, #40877, #16513, .T. ) ;
#123461=VECTOR ( 'NONE', #57737, 1000.000000000000000 ) ;
#123462=CIRCLE ( 'NONE', #50324, 0.1000000000000002554 ) ;
#123463=DIRECTION ( 'NONE',  ( -0.000000000000000000, -1.000000000000000000, -0.000000000000000000 ) ) ;
#123465=ORIENTED_EDGE ( 'NONE', *, *, #97307, .T. ) ;
#123466=ORIENTED_EDGE ( 'NONE', *, *, #86781, .F. ) ;
#123467=EDGE_LOOP ( 'NONE', ( #59800, #11952, #4847, #108707 ) ) ;
#123468=ORIENTED_EDGE ( 'NONE', *, *, #90089, .T. ) ;
#123469=ORIENTED_EDGE ( 'NONE', *, *, #93707, .T. ) ;
#123470=DIRECTION ( 'NONE',  ( -0.000000000000000000, 1.000000000000000000, -0.000000000000000000 ) ) ;
#123471=DIRECTION ( 'NONE',  ( 0.000000000000000000, -0.000000000000000000, 1.000000000000000000 ) ) ;
#123472=ORIENTED_EDGE ( 'NONE', *, *, #30656, .T. ) ;
#123473=ADVANCED_FACE ( 'NONE', ( #125919 ), #66703, .T. ) ;
#123474=FACE_BOUND ( 'NONE', #17904, .T. ) ;
#123475=CIRCLE ( 'NONE', #104691, 0.06509327318403745899 ) ;
#123476=CARTESIAN_POINT ( 'NONE',  ( -6.850000000000013856, 2.500000000000000000, 6.741600689897071952 ) ) ;
#123477=EDGE_CURVE ( 'NONE', #95827, #126422, #66362, .T. ) ;
#123478=EDGE_CURVE ( 'NONE', #53570, #61169, #89692, .T. ) ;
#123479=ADVANCED_FACE ( 'NONE', ( #97762 ), #83455, .T. ) ;
#123480=EDGE_LOOP ( 'NONE', ( #74790, #93304, #43959, #30461 ) ) ;
#123481=DIRECTION ( 'NONE',  ( 0.000000000000000000, 0.000000000000000000, 1.000000000000000000 ) ) ;
#123482=CARTESIAN_POINT ( 'NONE',  ( 4.599999999999935696, 2.500000000000000000, 5.122947341949749323 ) ) ;
#123483=DIRECTION ( 'NONE',  ( -4.274815082592931898E-19, -0.9999939076577903929, -0.003490651415223739937 ) ) ;
#123484=ORIENTED_EDGE ( 'NONE', *, *, #827, .F. ) ;
#123486=EDGE_CURVE ( 'NONE', #39021, #15192, #36922, .T. ) ;
#123487=CIRCLE ( 'NONE', #67040, 0.06509327318403745899 ) ;
#123488=VERTEX_POINT ( 'NONE', #78135 ) ;
#123489=CONICAL_SURFACE ( 'NONE', #29510, 0.09999999999999982514, 0.003490658503988666988 ) ;
#123490=EDGE_LOOP ( 'NONE', ( #74127, #111745 ) ) ;
#123491=ORIENTED_EDGE ( 'NONE', *, *, #90622, .F. ) ;
#123492=DIRECTION ( 'NONE',  ( -0.000000000000000000, -1.000000000000000000, -0.000000000000000000 ) ) ;
#123493=DIRECTION ( 'NONE',  ( 0.000000000000000000, 0.000000000000000000, 1.000000000000000000 ) ) ;
#123494=DIRECTION ( 'NONE',  ( 0.000000000000000000, 1.000000000000000000, 0.000000000000000000 ) ) ;
#123495=EDGE_LOOP ( 'NONE', ( #29439, #57288, #62312, #99592 ) ) ;
#123496=CARTESIAN_POINT ( 'NONE',  ( 10.39999999999991509, 2.500000000000000000, 0.7928203230275495672 ) ) ;
#123497=AXIS2_PLACEMENT_3D ( 'NONE', #17515, #99963, #60058 ) ;
#123498=DIRECTION ( 'NONE',  ( -0.000000000000000000, -1.000000000000000000, -0.000000000000000000 ) ) ;
#123499=CARTESIAN_POINT ( 'NONE',  ( -10.85000000000000142, 12.50000000000000000, -6.560283801567336148 ) ) ;
#123500=VECTOR ( 'NONE', #109643, 1000.000000000000000 ) ;
#123502=ORIENTED_EDGE ( 'NONE', *, *, #9948, .F. ) ;
#123503=LINE ( 'NONE', #64590, #87134 ) ;
#123504=EDGE_CURVE ( 'NONE', #27665, #106728, #121086, .T. ) ;
#123505=ORIENTED_EDGE ( 'NONE', *, *, #21427, .F. ) ;
#123506=DIRECTION ( 'NONE',  ( 0.000000000000000000, -0.000000000000000000, 1.000000000000000000 ) ) ;
#123507=ORIENTED_EDGE ( 'NONE', *, *, #18548, .T. ) ;
#123508=EDGE_LOOP ( 'NONE', ( #100606, #24469 ) ) ;
#123509=CARTESIAN_POINT ( 'NONE',  ( 8.549999999999922551, 12.50000000000000000, -6.148780366869526226 ) ) ;
#123510=DIRECTION ( 'NONE',  ( 0.000000000000000000, 0.000000000000000000, -1.000000000000000000 ) ) ;
#123511=DIRECTION ( 'NONE',  ( -0.000000000000000000, -1.000000000000000000, -0.000000000000000000 ) ) ;
#123512=FACE_OUTER_BOUND ( 'NONE', #125711, .T. ) ;
#123513=CARTESIAN_POINT ( 'NONE',  ( -14.54999999999998472, 2.500000000000000000, 2.265063509461101354 ) ) ;
#123514=ORIENTED_EDGE ( 'NONE', *, *, #121583, .T. ) ;
#123515=ORIENTED_EDGE ( 'NONE', *, *, #119492, .F. ) ;
#123516=FACE_OUTER_BOUND ( 'NONE', #6326, .T. ) ;
#123517=EDGE_CURVE ( 'NONE', #907, #63096, #37482, .T. ) ;
#123519=CIRCLE ( 'NONE', #75405, 0.09999999999999999167 ) ;
#123520=DIRECTION ( 'NONE',  ( -0.000000000000000000, -1.000000000000000000, -0.000000000000000000 ) ) ;
#123521=ORIENTED_EDGE ( 'NONE', *, *, #83085, .T. ) ;
#123522=ORIENTED_EDGE ( 'NONE', *, *, #30963, .F. ) ;
#123523=AXIS2_PLACEMENT_3D ( 'NONE', #74791, #114696, #55789 ) ;
#123524=VECTOR ( 'NONE', #61246, 1000.000000000000000 ) ;
#123525=DIRECTION ( 'NONE',  ( 0.000000000000000000, 1.000000000000000000, 0.000000000000000000 ) ) ;
#123526=ORIENTED_EDGE ( 'NONE', *, *, #91780, .F. ) ;
#123527=DIRECTION ( 'NONE',  ( 0.000000000000000000, 1.000000000000000000, 0.000000000000000000 ) ) ;
#123528=CIRCLE ( 'NONE', #31512, 0.09999999999999982514 ) ;
#123530=VERTEX_POINT ( 'NONE', #129192 ) ;
#123531=DIRECTION ( 'NONE',  ( 0.000000000000000000, 0.000000000000000000, 1.000000000000000000 ) ) ;
#123532=DIRECTION ( 'NONE',  ( 0.000000000000000000, 0.000000000000000000, -1.000000000000000000 ) ) ;
#123533=DIRECTION ( 'NONE',  ( 0.000000000000000000, 1.000000000000000000, 0.000000000000000000 ) ) ;
#123534=CIRCLE ( 'NONE', #58704, 0.1000000000000002554 ) ;
#123535=EDGE_CURVE ( 'NONE', #19955, #68062, #110167, .T. ) ;
#123537=EDGE_LOOP ( 'NONE', ( #3227, #47578 ) ) ;
#123538=DIRECTION ( 'NONE',  ( 0.000000000000000000, 0.000000000000000000, -1.000000000000000000 ) ) ;
#123539=CARTESIAN_POINT ( 'NONE',  ( 21.15177371151419550, -2.593223176056363766, 4.151029080743462885 ) ) ;
#123540=EDGE_LOOP ( 'NONE', ( #16820, #94731, #1101, #26837 ) ) ;
#123541=ORIENTED_EDGE ( 'NONE', *, *, #88568, .F. ) ;
#123543=CARTESIAN_POINT ( 'NONE',  ( -4.600000000000028955, 2.500000000000000000, -4.330127018922201643 ) ) ;
#123544=DIRECTION ( 'NONE',  ( -0.000000000000000000, 1.000000000000000000, -0.000000000000000000 ) ) ;
#123545=CARTESIAN_POINT ( 'NONE',  ( -3.750000000000026201, 2.500000000000000000, 5.702370205355745014 ) ) ;
#123546=LINE ( 'NONE', #71901, #100825 ) ;
#123547=LINE ( 'NONE', #14238, #88943 ) ;
#123548=CARTESIAN_POINT ( 'NONE',  ( 14.59999999999989484, 12.50000000000000000, 0.6277270498435120194 ) ) ;
#123549=CARTESIAN_POINT ( 'NONE',  ( -4.293440603042597559E-14, 12.50000000000000000, 5.088040615133786027 ) ) ;
#123550=DIRECTION ( 'NONE',  ( 0.000000000000000000, -0.9999939076577903929, 0.003490651415223739937 ) ) ;
#123551=DIRECTION ( 'NONE',  ( -0.000000000000000000, -1.000000000000000000, -0.000000000000000000 ) ) ;
#123552=CARTESIAN_POINT ( 'NONE',  ( 3.349999999999941025, 2.500000000000000000, 7.288010851410849256 ) ) ;
#123553=AXIS2_PLACEMENT_3D ( 'NONE', #66091, #16957, #67353 ) ;
#123554=ORIENTED_EDGE ( 'NONE', *, *, #104392, .T. ) ;
#123555=AXIS2_PLACEMENT_3D ( 'NONE', #69124, #9575, #20686 ) ;
#123556=VERTEX_POINT ( 'NONE', #50588 ) ;
#123558=ORIENTED_EDGE ( 'NONE', *, *, #96445, .T. ) ;
#123560=DIRECTION ( 'NONE',  ( 0.000000000000000000, -0.000000000000000000, 1.000000000000000000 ) ) ;
#123561=DIRECTION ( 'NONE',  ( 0.000000000000000000, 0.000000000000000000, 1.000000000000000000 ) ) ;
#123562=VECTOR ( 'NONE', #103815, 1000.000000000000000 ) ;
#123563=EDGE_CURVE ( 'NONE', #95146, #61052, #22989, .T. ) ;
#123564=CIRCLE ( 'NONE', #77596, 0.1000000000000002554 ) ;
#123565=ORIENTED_EDGE ( 'NONE', *, *, #46765, .T. ) ;
#123566=DIRECTION ( 'NONE',  ( 0.000000000000000000, 0.000000000000000000, -1.000000000000000000 ) ) ;
#123567=CARTESIAN_POINT ( 'NONE',  ( -6.700000000000016165, 2.500000000000000000, 4.430127018922196847 ) ) ;
#123569=VERTEX_POINT ( 'NONE', #11315 ) ;
#123570=EDGE_CURVE ( 'NONE', #73695, #97932, #6229, .T. ) ;
#123571=ADVANCED_FACE ( 'NONE', ( #19857 ), #58507, .T. ) ;
#123572=EDGE_CURVE ( 'NONE', #20221, #72457, #10640, .T. ) ;
#123573=FACE_OUTER_BOUND ( 'NONE', #14555, .T. ) ;
#123574=EDGE_CURVE ( 'NONE', #51919, #54631, #108652, .T. ) ;
#123575=DIRECTION ( 'NONE',  ( 0.000000000000000000, -0.000000000000000000, 1.000000000000000000 ) ) ;
#123576=CONICAL_SURFACE ( 'NONE', #86002, 0.1000000000000000056, 0.003490658503988666988 ) ;
#123577=EDGE_LOOP ( 'NONE', ( #28291, #94575 ) ) ;
#123578=CONICAL_SURFACE ( 'NONE', #67120, 0.1000000000000000056, 0.003490658503988666988 ) ;
#123579=ORIENTED_EDGE ( 'NONE', *, *, #16743, .T. ) ;
#123580=ORIENTED_EDGE ( 'NONE', *, *, #44518, .T. ) ;
#123581=ORIENTED_EDGE ( 'NONE', *, *, #50040, .T. ) ;
#123582=LINE ( 'NONE', #63391, #67742 ) ;
#123583=EDGE_CURVE ( 'NONE', #81003, #27779, #121177, .T. ) ;
#123584=AXIS2_PLACEMENT_3D ( 'NONE', #41063, #33790, #52783 ) ;
#123585=DIRECTION ( 'NONE',  ( 0.000000000000000000, 1.000000000000000000, 0.000000000000000000 ) ) ;
#123586=CARTESIAN_POINT ( 'NONE',  ( 2.500000000000002220, -1.761799387799150018, -9.999999999999998224 ) ) ;
#123587=ADVANCED_FACE ( 'NONE', ( #29041 ), #91938, .T. ) ;
#123589=EDGE_CURVE ( 'NONE', #33696, #7764, #35517, .T. ) ;
#123590=VERTEX_POINT ( 'NONE', #80716 ) ;
#123591=AXIS2_PLACEMENT_3D ( 'NONE', #116711, #88543, #37532 ) ;
#123592=CIRCLE ( 'NONE', #6490, 0.09999999999999982514 ) ;
#123593=CARTESIAN_POINT ( 'NONE',  ( 8.549999999999920774, 12.50000000000000000, -2.511473670974877948 ) ) ;
#123594=ORIENTED_EDGE ( 'NONE', *, *, #29629, .F. ) ;
#123596=DIRECTION ( 'NONE',  ( 0.000000000000000000, 0.000000000000000000, 1.000000000000000000 ) ) ;
#123597=CARTESIAN_POINT ( 'NONE',  ( -14.79999999999998295, 2.500000000000000000, -0.3464101615137760715 ) ) ;
#123598=ORIENTED_EDGE ( 'NONE', *, *, #109566, .F. ) ;
#123599=ORIENTED_EDGE ( 'NONE', *, *, #121424, .T. ) ;
#123600=ORIENTED_EDGE ( 'NONE', *, *, #116734, .F. ) ;
#123601=DIRECTION ( 'NONE',  ( -0.000000000000000000, 1.000000000000000000, -0.000000000000000000 ) ) ;
#123602=CARTESIAN_POINT ( 'NONE',  ( 12.89999999999989910, 2.500000000000000000, 0.6928203230275494784 ) ) ;
#123603=DIRECTION ( 'NONE',  ( 0.000000000000000000, 0.000000000000000000, 1.000000000000000000 ) ) ;
#123604=FACE_BOUND ( 'NONE', #3926, .T. ) ;
#123605=CARTESIAN_POINT ( 'NONE',  ( -8.749999999999975131, 2.500000000000000000, 2.165063509461097713 ) ) ;
#123606=PLANE ( 'NONE',  #44444 ) ;
#123607=DIRECTION ( 'NONE',  ( 0.000000000000000000, 0.000000000000000000, 1.000000000000000000 ) ) ;
#123608=CONICAL_SURFACE ( 'NONE', #102683, 0.09999999999999982514, 0.003490658503988666988 ) ;
#123609=CIRCLE ( 'NONE', #96416, 0.06509327318403743123 ) ;
#123610=DIRECTION ( 'NONE',  ( 0.000000000000000000, 0.000000000000000000, 1.000000000000000000 ) ) ;
#123611=VECTOR ( 'NONE', #32942, 1000.000000000000000 ) ;
#123612=CARTESIAN_POINT ( 'NONE',  ( 12.09999999999990550, 12.50000000000000000, 5.088040615133786027 ) ) ;
#123613=CARTESIAN_POINT ( 'NONE',  ( 0.6499999999999543920, 2.500000000000000000, 6.841600689897072485 ) ) ;
#123614=EDGE_LOOP ( 'NONE', ( #122282, #117305 ) ) ;
#123615=CONICAL_SURFACE ( 'NONE', #42077, 0.1000000000000002554, 0.003490658503988666988 ) ;
#123616=DIRECTION ( 'NONE',  ( -0.000000000000000000, -1.000000000000000000, -0.000000000000000000 ) ) ;
#123617=ORIENTED_EDGE ( 'NONE', *, *, #12576, .T. ) ;
#123618=ORIENTED_EDGE ( 'NONE', *, *, #102751, .F. ) ;
#123619=EDGE_LOOP ( 'NONE', ( #86318, #80906, #108739, #19288 ) ) ;
#123620=VERTEX_POINT ( 'NONE', #109522 ) ;
#123621=AXIS2_PLACEMENT_3D ( 'NONE', #5510, #46103, #93918 ) ;
#123622=DIRECTION ( 'NONE',  ( 0.000000000000000000, -0.9999939076577903929, 0.003490651415223739937 ) ) ;
#123623=EDGE_CURVE ( 'NONE', #98683, #18231, #70244, .T. ) ;
#123624=FACE_BOUND ( 'NONE', #25097, .T. ) ;
#123625=DIRECTION ( 'NONE',  ( 0.000000000000000000, 0.000000000000000000, -1.000000000000000000 ) ) ;
#123626=EDGE_CURVE ( 'NONE', #98794, #88843, #100351, .T. ) ;
#123628=EDGE_LOOP ( 'NONE', ( #103262, #30410 ) ) ;
#123629=CARTESIAN_POINT ( 'NONE',  ( -12.89999999999999147, 2.500000000000000000, -5.022947341949751454 ) ) ;
#123630=LINE ( 'NONE', #33982, #52012 ) ;
#123631=ORIENTED_EDGE ( 'NONE', *, *, #98264, .F. ) ;
#123632=FACE_OUTER_BOUND ( 'NONE', #85381, .T. ) ;
#123633=DIRECTION ( 'NONE',  ( 0.000000000000000000, 0.000000000000000000, -1.000000000000000000 ) ) ;
#123634=EDGE_CURVE ( 'NONE', #93851, #114560, #66784, .T. ) ;
#123635=ORIENTED_EDGE ( 'NONE', *, *, #115816, .F. ) ;
#123636=DIRECTION ( 'NONE',  ( 0.000000000000000000, -0.000000000000000000, 1.000000000000000000 ) ) ;
#123637=DIRECTION ( 'NONE',  ( 0.000000000000000000, 0.000000000000000000, 1.000000000000000000 ) ) ;
#123638=ORIENTED_EDGE ( 'NONE', *, *, #27649, .F. ) ;
#123639=DIRECTION ( 'NONE',  ( -4.274815082592931898E-19, -0.9999939076577903929, -0.003490651415223739937 ) ) ;
#123640=DIRECTION ( 'NONE',  ( -0.000000000000000000, 1.000000000000000000, -0.000000000000000000 ) ) ;
#123641=CARTESIAN_POINT ( 'NONE',  ( -11.04999999999999893, 2.500000000000000000, 6.148780366869520009 ) ) ;
#123642=ORIENTED_EDGE ( 'NONE', *, *, #59657, .F. ) ;
#123643=EDGE_LOOP ( 'NONE', ( #10193, #111151 ) ) ;
#123644=CARTESIAN_POINT ( 'NONE',  ( -1.050000000000037348, 2.500000000000000000, -2.611473670974877592 ) ) ;
#123645=ADVANCED_FACE ( 'NONE', ( #68291 ), #41447, .T. ) ;
#123646=CIRCLE ( 'NONE', #111126, 0.1000000000000002554 ) ;
#123647=ORIENTED_EDGE ( 'NONE', *, *, #76299, .F. ) ;
#123648=CARTESIAN_POINT ( 'NONE',  ( -1.700000000000035261, 2.500000000000000000, 4.430127018922196847 ) ) ;
#123649=CIRCLE ( 'NONE', #56741, 0.06509327318403745899 ) ;
#123650=CARTESIAN_POINT ( 'NONE',  ( 12.49999999999990408, 12.50000000000000000, 5.022947341949748790 ) ) ;
#123651=ORIENTED_EDGE ( 'NONE', *, *, #82837, .T. ) ;
#123652=CIRCLE ( 'NONE', #27803, 0.06509327318403745899 ) ;
#123653=CARTESIAN_POINT ( 'NONE',  ( -6.900000000000019007, 2.500000000000000000, 0.4464101615137735513 ) ) ;
#123654=CARTESIAN_POINT ( 'NONE',  ( -0.6500000000000394351, 12.50000000000000000, 6.841600689897072485 ) ) ;
#123655=CARTESIAN_POINT ( 'NONE',  ( -4.800000000000026468, 12.50000000000000000, -4.611443907251940644 ) ) ;
#123656=LINE ( 'NONE', #16277, #96663 ) ;
#123657=FACE_OUTER_BOUND ( 'NONE', #94411, .T. ) ;
#123658=VECTOR ( 'NONE', #126671, 1000.000000000000000 ) ;
#123659=ORIENTED_EDGE ( 'NONE', *, *, #109624, .F. ) ;
#123660=VERTEX_POINT ( 'NONE', #24365 ) ;
#123662=EDGE_CURVE ( 'NONE', #52089, #92128, #85668, .T. ) ;
#123664=VERTEX_POINT ( 'NONE', #2784 ) ;
#123665=ORIENTED_EDGE ( 'NONE', *, *, #33148, .F. ) ;
#123666=ORIENTED_EDGE ( 'NONE', *, *, #12308, .T. ) ;
#123667=DIRECTION ( 'NONE',  ( 0.000000000000000000, 0.000000000000000000, 1.000000000000000000 ) ) ;
#123668=CIRCLE ( 'NONE', #63054, 0.1000000000000002554 ) ;
#123669=DIRECTION ( 'NONE',  ( -0.000000000000000000, 1.000000000000000000, -0.000000000000000000 ) ) ;
#123672=DIRECTION ( 'NONE',  ( -1.000000000000000000, -0.000000000000000000, -0.000000000000000000 ) ) ;
#123673=AXIS2_PLACEMENT_3D ( 'NONE', #73410, #61686, #52482 ) ;
#123674=AXIS2_PLACEMENT_3D ( 'NONE', #101178, #41638, #81537 ) ;
#123675=CARTESIAN_POINT ( 'NONE',  ( 7.099999999999926814, 2.500000000000000000, -0.1000000000000022815 ) ) ;
#123676=DIRECTION ( 'NONE',  ( 0.000000000000000000, 0.000000000000000000, -1.000000000000000000 ) ) ;
#123677=DIRECTION ( 'NONE',  ( 0.000000000000000000, 0.000000000000000000, 1.000000000000000000 ) ) ;
#123678=DIRECTION ( 'NONE',  ( 0.000000000000000000, 0.000000000000000000, 1.000000000000000000 ) ) ;
#123679=ADVANCED_FACE ( 'NONE', ( #104205 ), #94377, .T. ) ;
#123680=CARTESIAN_POINT ( 'NONE',  ( 2.299999999999948752, 2.500000000000000000, 0.3464101615137735735 ) ) ;
#123681=VERTEX_POINT ( 'NONE', #42744 ) ;
#123682=CARTESIAN_POINT ( 'NONE',  ( 4.799999999999935874, 12.50000000000000000, 3.983716857408420964 ) ) ;
#123683=EDGE_LOOP ( 'NONE', ( #50201, #35805 ) ) ;
#123684=EDGE_CURVE ( 'NONE', #63642, #105966, #52239, .T. ) ;
#123685=EDGE_LOOP ( 'NONE', ( #88266, #30884 ) ) ;
#123686=DIRECTION ( 'NONE',  ( 0.000000000000000000, 0.000000000000000000, -1.000000000000000000 ) ) ;
#123687=LINE ( 'NONE', #95548, #23845 ) ;
#123688=CARTESIAN_POINT ( 'NONE',  ( 12.69999999999989804, 12.50000000000000000, 0.2813168883297361700 ) ) ;
#123689=DIRECTION ( 'NONE',  ( 0.000000000000000000, 0.000000000000000000, -1.000000000000000000 ) ) ;
#123690=CARTESIAN_POINT ( 'NONE',  ( -1.850000000000033840, 12.50000000000000000, 6.906693963081109722 ) ) ;
#123691=DIRECTION ( 'NONE',  ( 0.000000000000000000, 1.000000000000000000, 0.000000000000000000 ) ) ;
#123692=VECTOR ( 'NONE', #3219, 1000.000000000000000 ) ;
#123693=CARTESIAN_POINT ( 'NONE',  ( -7.900000000000011013, 12.50000000000000000, 4.330127018922196314 ) ) ;
#123694=EDGE_LOOP ( 'NONE', ( #122743, #72873 ) ) ;
#123695=DIRECTION ( 'NONE',  ( 0.000000000000000000, 0.000000000000000000, 1.000000000000000000 ) ) ;
#123696=CIRCLE ( 'NONE', #44289, 0.06509327318403745899 ) ;
#123697=AXIS2_PLACEMENT_3D ( 'NONE', #24388, #64303, #104233 ) ;
#123698=DIRECTION ( 'NONE',  ( -0.000000000000000000, -1.000000000000000000, -0.000000000000000000 ) ) ;
#123699=ORIENTED_EDGE ( 'NONE', *, *, #45471, .T. ) ;
#123700=VECTOR ( 'NONE', #33317, 1000.000000000000000 ) ;
#123701=VERTEX_POINT ( 'NONE', #2134 ) ;
#123702=EDGE_CURVE ( 'NONE', #64648, #62406, #20841, .T. ) ;
#123703=ORIENTED_EDGE ( 'NONE', *, *, #104388, .F. ) ;
#123705=CIRCLE ( 'NONE', #88193, 0.1000000000000002554 ) ;
#123706=ORIENTED_EDGE ( 'NONE', *, *, #5425, .T. ) ;
#123707=DIRECTION ( 'NONE',  ( -4.274815082592931898E-19, -0.9999939076577903929, -0.003490651415223739937 ) ) ;
#123708=CARTESIAN_POINT ( 'NONE',  ( 8.099999999999923261, 2.500000000000000000, 3.983716857408420076 ) ) ;
#123709=AXIS2_PLACEMENT_3D ( 'NONE', #75031, #4323, #73724 ) ;
#123710=EDGE_CURVE ( 'NONE', #90525, #48509, #79436, .T. ) ;
#123711=CARTESIAN_POINT ( 'NONE',  ( 11.64999999999990798, 12.50000000000000000, 5.802370205355744659 ) ) ;
#123712=CARTESIAN_POINT ( 'NONE',  ( -1.650000000000034328, 2.500000000000000000, -2.165063509461101710 ) ) ;
#123713=DIRECTION ( 'NONE',  ( 0.000000000000000000, -0.9999939076577903929, 0.003490651415223739937 ) ) ;
#123714=ORIENTED_EDGE ( 'NONE', *, *, #21225, .T. ) ;
#123715=CARTESIAN_POINT ( 'NONE',  ( -10.65000000000000213, 2.500000000000000000, 1.918653347947321564 ) ) ;
#123716=ADVANCED_FACE ( 'NONE', ( #82649 ), #12504, .T. ) ;
#123718=EDGE_CURVE ( 'NONE', #113976, #27106, #93992, .T. ) ;
#123719=CARTESIAN_POINT ( 'NONE',  ( -5.850000000000022737, 2.500000000000000000, -2.165063509461101710 ) ) ;
#123721=DIRECTION ( 'NONE',  ( 0.000000000000000000, 0.000000000000000000, 1.000000000000000000 ) ) ;
#123722=ORIENTED_EDGE ( 'NONE', *, *, #103648, .F. ) ;
#123723=ORIENTED_EDGE ( 'NONE', *, *, #19830, .T. ) ;
#123724=ADVANCED_FACE ( 'NONE', ( #54456 ), #51901, .T. ) ;
#123725=EDGE_LOOP ( 'NONE', ( #56850, #19737 ) ) ;
#123726=DIRECTION ( 'NONE',  ( 0.000000000000000000, 0.000000000000000000, -1.000000000000000000 ) ) ;
#123727=ADVANCED_FACE ( 'NONE', ( #122570 ), #12592, .T. ) ;
#123728=CARTESIAN_POINT ( 'NONE',  ( -11.05000000000000249, 2.500000000000000000, -6.248780366869523206 ) ) ;
#123729=CIRCLE ( 'NONE', #42284, 0.1000000000000002554 ) ;
#123731=VECTOR ( 'NONE', #91849, 1000.000000000000000 ) ;
#123732=ADVANCED_FACE ( 'NONE', ( #11955 ), #45982, .T. ) ;
#123733=EDGE_CURVE ( 'NONE', #39644, #4240, #18767, .T. ) ;
#123734=ORIENTED_EDGE ( 'NONE', *, *, #99248, .F. ) ;
#123735=DIRECTION ( 'NONE',  ( -0.000000000000000000, -1.000000000000000000, -0.000000000000000000 ) ) ;
#123736=CARTESIAN_POINT ( 'NONE',  ( 6.899999999999928413, 12.50000000000000000, 3.918623584224383727 ) ) ;
#123737=DIRECTION ( 'NONE',  ( 0.000000000000000000, 1.000000000000000000, 0.000000000000000000 ) ) ;
#123738=FACE_OUTER_BOUND ( 'NONE', #97733, .T. ) ;
#123739=AXIS2_PLACEMENT_3D ( 'NONE', #61963, #13481, #92708 ) ;
#123740=EDGE_CURVE ( 'NONE', #96862, #33099, #100259, .T. ) ;
#123741=CONICAL_SURFACE ( 'NONE', #52654, 0.1000000000000000472, 0.003490658503988666988 ) ;
#123742=AXIS2_PLACEMENT_3D ( 'NONE', #116636, #75421, #115324 ) ;
#123743=CARTESIAN_POINT ( 'NONE',  ( 14.14999999999989555, 2.500000000000000000, 2.165063509461097713 ) ) ;
#123744=CIRCLE ( 'NONE', #10866, 0.1000000000000000472 ) ;
#123745=EDGE_LOOP ( 'NONE', ( #28781, #123469, #52387, #117109 ) ) ;
#123746=ORIENTED_EDGE ( 'NONE', *, *, #62734, .F. ) ;
#123747=LINE ( 'NONE', #74027, #81474 ) ;
#123748=DIRECTION ( 'NONE',  ( 0.000000000000000000, 0.000000000000000000, 1.000000000000000000 ) ) ;
#123749=DIRECTION ( 'NONE',  ( 0.000000000000000000, 0.000000000000000000, 1.000000000000000000 ) ) ;
#123750=AXIS2_PLACEMENT_3D ( 'NONE', #24932, #70329, #4607 ) ;
#123751=FACE_OUTER_BOUND ( 'NONE', #75319, .T. ) ;
#123753=DIRECTION ( 'NONE',  ( -0.000000000000000000, -1.000000000000000000, -0.000000000000000000 ) ) ;
#123754=VERTEX_POINT ( 'NONE', #62994 ) ;
#123755=CIRCLE ( 'NONE', #10861, 0.06509327318403745899 ) ;
#123756=CIRCLE ( 'NONE', #48471, 0.06509327318403743123 ) ;
#123757=AXIS2_PLACEMENT_3D ( 'NONE', #4050, #53801, #71506 ) ;
#123758=ORIENTED_EDGE ( 'NONE', *, *, #64492, .F. ) ;
#123759=DIRECTION ( 'NONE',  ( 0.000000000000000000, 0.000000000000000000, 1.000000000000000000 ) ) ;
#123760=CARTESIAN_POINT ( 'NONE',  ( 8.149999999999923972, 2.500000000000000000, 2.611473670974873151 ) ) ;
#123761=CARTESIAN_POINT ( 'NONE',  ( 3.149999999999944400, 12.50000000000000000, 2.511473670974873507 ) ) ;
#123762=CIRCLE ( 'NONE', #52684, 0.06509327318403745899 ) ;
#123763=DIRECTION ( 'NONE',  ( 0.000000000000000000, 0.000000000000000000, -1.000000000000000000 ) ) ;
#123764=ORIENTED_EDGE ( 'NONE', *, *, #23724, .F. ) ;
#123765=DIRECTION ( 'NONE',  ( -0.000000000000000000, 1.000000000000000000, -0.000000000000000000 ) ) ;
#123766=DIRECTION ( 'NONE',  ( 0.000000000000000000, 0.000000000000000000, 1.000000000000000000 ) ) ;
#123767=AXIS2_PLACEMENT_3D ( 'NONE', #25590, #58945, #117832 ) ;
#123768=ORIENTED_EDGE ( 'NONE', *, *, #41777, .T. ) ;
#123769=CARTESIAN_POINT ( 'NONE',  ( -2.900000000000030109, 12.50000000000000000, 0.6928203230275494784 ) ) ;
#123770=EDGE_LOOP ( 'NONE', ( #11590, #61601 ) ) ;
#123771=DIRECTION ( 'NONE',  ( -0.000000000000000000, -1.000000000000000000, -0.000000000000000000 ) ) ;
#123772=ADVANCED_FACE ( 'NONE', ( #112750 ), #102407, .T. ) ;
#123773=ORIENTED_EDGE ( 'NONE', *, *, #74344, .T. ) ;
#123774=DIRECTION ( 'NONE',  ( 0.000000000000000000, 1.000000000000000000, 0.000000000000000000 ) ) ;
#123775=FACE_OUTER_BOUND ( 'NONE', #94573, .T. ) ;
#123776=EDGE_CURVE ( 'NONE', #71314, #102506, #101642, .T. ) ;
#123777=VERTEX_POINT ( 'NONE', #114034 ) ;
#123778=ORIENTED_EDGE ( 'NONE', *, *, #40246, .T. ) ;
#123780=DIRECTION ( 'NONE',  ( 0.000000000000000000, 1.000000000000000000, 0.000000000000000000 ) ) ;
#123782=CARTESIAN_POINT ( 'NONE',  ( -12.94999999999999218, 2.500000000000000000, -2.165063509461099489 ) ) ;
#123783=EDGE_CURVE ( 'NONE', #103364, #104181, #25570, .T. ) ;
#123784=AXIS2_PLACEMENT_3D ( 'NONE', #60065, #51520, #70499 ) ;
#123785=DIRECTION ( 'NONE',  ( 0.000000000000000000, 0.000000000000000000, -1.000000000000000000 ) ) ;
#123786=DIRECTION ( 'NONE',  ( -4.274815082592931898E-19, -0.9999939076577903929, -0.003490651415223739937 ) ) ;
#123788=AXIS2_PLACEMENT_3D ( 'NONE', #47902, #98919, #68164 ) ;
#123789=CARTESIAN_POINT ( 'NONE',  ( -1.650000000000034328, 12.50000000000000000, -2.165063509461101710 ) ) ;
#123790=CARTESIAN_POINT ( 'NONE',  ( 9.549999999999915445, 2.500000000000000000, -2.265063509461101798 ) ) ;
#123791=VECTOR ( 'NONE', #26057, 1000.000000000000000 ) ;
#123792=AXIS2_PLACEMENT_3D ( 'NONE', #5873, #97496, #87027 ) ;
#123793=VERTEX_POINT ( 'NONE', #34784 ) ;
#123794=AXIS2_PLACEMENT_3D ( 'NONE', #9235, #89087, #69425 ) ;
#123795=ORIENTED_EDGE ( 'NONE', *, *, #101946, .T. ) ;
#123796=DIRECTION ( 'NONE',  ( -0.000000000000000000, 1.000000000000000000, -0.000000000000000000 ) ) ;
#123797=ORIENTED_EDGE ( 'NONE', *, *, #48023, .T. ) ;
#123798=DIRECTION ( 'NONE',  ( -0.000000000000000000, 1.000000000000000000, -0.000000000000000000 ) ) ;
#123799=DIRECTION ( 'NONE',  ( 0.000000000000000000, 0.000000000000000000, 1.000000000000000000 ) ) ;
#123800=AXIS2_PLACEMENT_3D ( 'NONE', #126583, #99056, #49331 ) ;
#123801=DIRECTION ( 'NONE',  ( -4.274815082592931898E-19, -0.9999939076577903929, -0.003490651415223739937 ) ) ;
#123802=AXIS2_PLACEMENT_3D ( 'NONE', #75232, #125609, #18245 ) ;
#123803=ORIENTED_EDGE ( 'NONE', *, *, #83244, .T. ) ;
#123804=EDGE_LOOP ( 'NONE', ( #63757, #126399, #116883, #43924 ) ) ;
#123805=DIRECTION ( 'NONE',  ( 0.000000000000000000, 1.000000000000000000, 0.000000000000000000 ) ) ;
#123806=ORIENTED_EDGE ( 'NONE', *, *, #18506, .F. ) ;
#123807=DIRECTION ( 'NONE',  ( 0.000000000000000000, 0.000000000000000000, 1.000000000000000000 ) ) ;
#123808=DIRECTION ( 'NONE',  ( 0.000000000000000000, 0.000000000000000000, 1.000000000000000000 ) ) ;
#123809=VECTOR ( 'NONE', #24723, 1000.000000000000000 ) ;
#123810=VERTEX_POINT ( 'NONE', #94981 ) ;
#123811=CARTESIAN_POINT ( 'NONE',  ( 4.799999999999935874, 12.50000000000000000, 0.2813168883297361700 ) ) ;
#123812=CARTESIAN_POINT ( 'NONE',  ( -9.600000000000008527, 2.500000000000000000, 0.09999999999999761857 ) ) ;
#123813=CARTESIAN_POINT ( 'NONE',  ( -9.600000000000008527, 2.500000000000000000, -4.430127018922197735 ) ) ;
#123814=DIRECTION ( 'NONE',  ( 0.000000000000000000, 0.000000000000000000, -1.000000000000000000 ) ) ;
#123816=CARTESIAN_POINT ( 'NONE',  ( 11.89999999999990443, 2.500000000000000000, 0.2464101615137736789 ) ) ;
#123818=CARTESIAN_POINT ( 'NONE',  ( 4.799999999999935874, 12.50000000000000000, 3.918623584224383727 ) ) ;
#123819=CARTESIAN_POINT ( 'NONE',  ( 1.649999999999951950, 2.500000000000000000, -7.188010851410854052 ) ) ;
#123820=CIRCLE ( 'NONE', #124111, 0.06509327318403743123 ) ;
#123821=EDGE_CURVE ( 'NONE', #35207, #54453, #87715, .T. ) ;
#123822=ORIENTED_EDGE ( 'NONE', *, *, #15628, .F. ) ;
#123823=ORIENTED_EDGE ( 'NONE', *, *, #38796, .T. ) ;
#123824=ORIENTED_EDGE ( 'NONE', *, *, #45936, .T. ) ;
#123825=FACE_OUTER_BOUND ( 'NONE', #6800, .T. ) ;
#123826=ORIENTED_EDGE ( 'NONE', *, *, #126434, .T. ) ;
#123827=ORIENTED_EDGE ( 'NONE', *, *, #76362, .F. ) ;
#123828=VERTEX_POINT ( 'NONE', #45884 ) ;
#123829=EDGE_LOOP ( 'NONE', ( #26817, #112143, #79215, #16536 ) ) ;
#123830=CARTESIAN_POINT ( 'NONE',  ( -10.65000000000000213, 2.500000000000000000, 6.248780366869520542 ) ) ;
#123831=AXIS2_PLACEMENT_3D ( 'NONE', #49396, #10709, #61130 ) ;
#123832=AXIS2_PLACEMENT_3D ( 'NONE', #2986, #111652, #70433 ) ;
#123833=FACE_OUTER_BOUND ( 'NONE', #17197, .T. ) ;
#123836=EDGE_CURVE ( 'NONE', #10045, #121533, #112870, .T. ) ;
#123837=DIRECTION ( 'NONE',  ( 0.000000000000000000, 0.000000000000000000, 1.000000000000000000 ) ) ;
#123838=EDGE_CURVE ( 'NONE', #105977, #34711, #2038, .T. ) ;
#123839=ORIENTED_EDGE ( 'NONE', *, *, #6121, .F. ) ;
#123840=AXIS2_PLACEMENT_3D ( 'NONE', #34445, #35719, #83539 ) ;
#123841=AXIS2_PLACEMENT_3D ( 'NONE', #120649, #19878, #99730 ) ;
#123842=CARTESIAN_POINT ( 'NONE',  ( -12.94999999999999218, 2.500000000000000000, 2.165063509461101265 ) ) ;
#123843=EDGE_LOOP ( 'NONE', ( #20435, #60359 ) ) ;
#123844=ORIENTED_EDGE ( 'NONE', *, *, #105709, .T. ) ;
#123845=AXIS2_PLACEMENT_3D ( 'NONE', #86714, #67046, #36975 ) ;
#123846=VERTEX_POINT ( 'NONE', #66149 ) ;
#123847=DIRECTION ( 'NONE',  ( 0.000000000000000000, 1.000000000000000000, 0.000000000000000000 ) ) ;
#123848=VERTEX_POINT ( 'NONE', #106085 ) ;
#123849=ADVANCED_FACE ( 'NONE', ( #26241 ), #56422, .T. ) ;
#123850=ORIENTED_EDGE ( 'NONE', *, *, #77078, .T. ) ;
#123851=ORIENTED_EDGE ( 'NONE', *, *, #11367, .F. ) ;
#123852=AXIS2_PLACEMENT_3D ( 'NONE', #96230, #117147, #86411 ) ;
#123853=CARTESIAN_POINT ( 'NONE',  ( -9.550000000000007816, 2.500000000000000000, -6.495190528383297135 ) ) ;
#123854=AXIS2_PLACEMENT_3D ( 'NONE', #29469, #79847, #35858 ) ;
#123855=DIRECTION ( 'NONE',  ( 0.000000000000000000, 0.000000000000000000, 1.000000000000000000 ) ) ;
#123856=CARTESIAN_POINT ( 'NONE',  ( -0.8500000000000386136, 12.50000000000000000, 1.472243186433545459 ) ) ;
#123857=DIRECTION ( 'NONE',  ( 0.000000000000000000, 1.000000000000000000, 0.000000000000000000 ) ) ;
#123858=VECTOR ( 'NONE', #126932, 1000.000000000000000 ) ;
#123859=CARTESIAN_POINT ( 'NONE',  ( 5.399999999999933742, 2.500000000000000000, -2.385244779468109755E-15 ) ) ;
#123860=AXIS2_PLACEMENT_3D ( 'NONE', #34041, #15010, #63509 ) ;
#123861=CIRCLE ( 'NONE', #126003, 0.06509327318403745899 ) ;
#123862=CARTESIAN_POINT ( 'NONE',  ( 16.56576425165007649, 1.499999999999997113, 6.084390597445792359 ) ) ;
#123863=AXIS2_PLACEMENT_3D ( 'NONE', #45733, #85643, #125559 ) ;
#123864=CARTESIAN_POINT ( 'NONE',  ( -8.150000000000009237, 2.500000000000000000, 6.841600689897072485 ) ) ;
#123865=EDGE_LOOP ( 'NONE', ( #41364, #52367 ) ) ;
#123866=FACE_OUTER_BOUND ( 'NONE', #98219, .T. ) ;
#123867=EDGE_LOOP ( 'NONE', ( #111010, #43589 ) ) ;
#123868=AXIS2_PLACEMENT_3D ( 'NONE', #122379, #121715, #120437 ) ;
#123869=DIRECTION ( 'NONE',  ( -0.000000000000000000, 1.000000000000000000, -0.000000000000000000 ) ) ;
#123870=ORIENTED_EDGE ( 'NONE', *, *, #74001, .F. ) ;
#123871=EDGE_LOOP ( 'NONE', ( #46979, #83955, #1854, #128107 ) ) ;
#123872=CARTESIAN_POINT ( 'NONE',  ( -1.050000000000038236, 2.500000000000000000, -6.148780366869526226 ) ) ;
#123874=ADVANCED_FACE ( 'NONE', ( #13820 ), #60650, .T. ) ;
#123875=DIRECTION ( 'NONE',  ( 0.000000000000000000, 0.000000000000000000, -1.000000000000000000 ) ) ;
#123876=ORIENTED_EDGE ( 'NONE', *, *, #103551, .F. ) ;
#123877=DIRECTION ( 'NONE',  ( 0.000000000000000000, -0.9999939076577903929, 0.003490651415223739937 ) ) ;
#123878=ORIENTED_EDGE ( 'NONE', *, *, #63218, .T. ) ;
#123879=CARTESIAN_POINT ( 'NONE',  ( 3.949999999999942446, 2.500000000000000000, -2.511473670974877948 ) ) ;
#123880=DIRECTION ( 'NONE',  ( 0.000000000000000000, 0.000000000000000000, -1.000000000000000000 ) ) ;
#123881=AXIS2_PLACEMENT_3D ( 'NONE', #4571, #36010, #75920 ) ;
#123882=EDGE_CURVE ( 'NONE', #41491, #116425, #56322, .T. ) ;
#123883=DIRECTION ( 'NONE',  ( 0.000000000000000000, 0.000000000000000000, -1.000000000000000000 ) ) ;
#123884=PLANE ( 'NONE',  #26251 ) ;
#123885=ADVANCED_FACE ( 'NONE', ( #56324 ), #39819, .T. ) ;
#123886=LINE ( 'NONE', #103626, #35489 ) ;
#123887=ORIENTED_EDGE ( 'NONE', *, *, #6761, .T. ) ;
#123888=CIRCLE ( 'NONE', #2604, 0.06509327318403743123 ) ;
#123889=CIRCLE ( 'NONE', #21501, 0.09999999999999982514 ) ;
#123890=EDGE_CURVE ( 'NONE', #23344, #30982, #10453, .T. ) ;
#123891=AXIS2_PLACEMENT_3D ( 'NONE', #102770, #13097, #53051 ) ;
#123892=EDGE_CURVE ( 'NONE', #34970, #118779, #6547, .T. ) ;
#123893=EDGE_CURVE ( 'NONE', #5233, #19176, #106595, .T. ) ;
#123894=VERTEX_POINT ( 'NONE', #84512 ) ;
#123895=DIRECTION ( 'NONE',  ( -0.000000000000000000, -1.000000000000000000, -0.000000000000000000 ) ) ;
#123896=DIRECTION ( 'NONE',  ( 0.000000000000000000, 1.000000000000000000, 0.000000000000000000 ) ) ;
#123897=VECTOR ( 'NONE', #5214, 1000.000000000000000 ) ;
#123898=CIRCLE ( 'NONE', #2614, 0.09999999999999982514 ) ;
#123899=AXIS2_PLACEMENT_3D ( 'NONE', #126643, #27147, #67043 ) ;
#123900=EDGE_CURVE ( 'NONE', #26093, #79044, #62793, .T. ) ;
#123901=CONICAL_SURFACE ( 'NONE', #111367, 0.1000000000000002554, 0.003490658503988666988 ) ;
#123903=CIRCLE ( 'NONE', #50763, 0.06509327318403741736 ) ;
#123905=LINE ( 'NONE', #94439, #111750 ) ;
#123906=CARTESIAN_POINT ( 'NONE',  ( 3.549999999999944755, 12.50000000000000000, -2.576566944158915184 ) ) ;
#123907=FACE_OUTER_BOUND ( 'NONE', #60204, .T. ) ;
#123908=DIRECTION ( 'NONE',  ( -0.000000000000000000, 1.000000000000000000, -0.000000000000000000 ) ) ;
#123909=ORIENTED_EDGE ( 'NONE', *, *, #114850, .F. ) ;
#123910=ADVANCED_FACE ( 'NONE', ( #113970 ), #69030, .T. ) ;
#123911=CIRCLE ( 'NONE', #2718, 0.06509327318403745899 ) ;
#123912=CARTESIAN_POINT ( 'NONE',  ( 1.649999999999950617, 2.500000000000000000, 2.165063509461097713 ) ) ;
#123913=FACE_OUTER_BOUND ( 'NONE', #30460, .T. ) ;
#123914=CARTESIAN_POINT ( 'NONE',  ( -4.400000000000025224, 2.500000000000000000, 4.676537180435972552 ) ) ;
#123915=ORIENTED_EDGE ( 'NONE', *, *, #103491, .T. ) ;
#123916=CARTESIAN_POINT ( 'NONE',  ( 5.399999999999932854, 2.500000000000000000, 3.737306695894644371 ) ) ;
#123917=AXIS2_PLACEMENT_3D ( 'NONE', #77552, #27812, #78224 ) ;
#123918=ORIENTED_EDGE ( 'NONE', *, *, #13676, .T. ) ;
#123919=CARTESIAN_POINT ( 'NONE',  ( 6.699999999999930012, 2.500000000000000000, -4.330127018922201643 ) ) ;
#123920=ORIENTED_EDGE ( 'NONE', *, *, #16223, .T. ) ;
#123921=CARTESIAN_POINT ( 'NONE',  ( -11.69999999999999929, 2.500000000000000000, 0.1000000000000017403 ) ) ;
#123922=CARTESIAN_POINT ( 'NONE',  ( -8.950000000000008171, 12.50000000000000000, -2.511473670974877948 ) ) ;
#123923=CARTESIAN_POINT ( 'NONE',  ( 4.549999999999935874, 2.500000000000000000, 6.495190528383297135 ) ) ;
#123924=ORIENTED_EDGE ( 'NONE', *, *, #95730, .T. ) ;
#123925=CIRCLE ( 'NONE', #80022, 0.06509327318403745899 ) ;
#123926=AXIS2_PLACEMENT_3D ( 'NONE', #62330, #31573, #3395 ) ;
#123927=CARTESIAN_POINT ( 'NONE',  ( 3.749999999999940492, 2.500000000000000000, 5.902370205355745192 ) ) ;
#123928=CARTESIAN_POINT ( 'NONE',  ( 5.199999999999933564, 2.500000000000000000, 0.3464101615137735735 ) ) ;
#123929=CONICAL_SURFACE ( 'NONE', #75816, 0.1000000000000002554, 0.003490658503988666988 ) ;
#123930=ORIENTED_EDGE ( 'NONE', *, *, #16592, .T. ) ;
#123931=CIRCLE ( 'NONE', #69561, 0.09999999999999982514 ) ;
#123932=CARTESIAN_POINT ( 'NONE',  ( -5.450000000000019718, 2.500000000000000000, 6.495190528383297135 ) ) ;
#123933=VECTOR ( 'NONE', #10559, 1000.000000000000000 ) ;
#123934=EDGE_CURVE ( 'NONE', #25872, #37345, #92024, .T. ) ;
#123936=ORIENTED_EDGE ( 'NONE', *, *, #120762, .T. ) ;
#123937=DIRECTION ( 'NONE',  ( 0.000000000000000000, 0.000000000000000000, 1.000000000000000000 ) ) ;
#123938=DIRECTION ( 'NONE',  ( 0.000000000000000000, 0.000000000000000000, -1.000000000000000000 ) ) ;
#123939=PLANE ( 'NONE',  #82014 ) ;
#123940=ORIENTED_EDGE ( 'NONE', *, *, #23131, .T. ) ;
#123941=DIRECTION ( 'NONE',  ( 0.000000000000000000, 0.000000000000000000, -1.000000000000000000 ) ) ;
#123942=CARTESIAN_POINT ( 'NONE',  ( -0.2000000000000412836, 2.500000000000000000, 4.676537180435972552 ) ) ;
#123943=CONICAL_SURFACE ( 'NONE', #2768, 0.09999999999999999167, 0.003490658503988666988 ) ;
#123944=ORIENTED_EDGE ( 'NONE', *, *, #95663, .F. ) ;
#123945=EDGE_CURVE ( 'NONE', #99630, #12428, #12596, .T. ) ;
#123946=DIRECTION ( 'NONE',  ( 0.000000000000000000, 0.000000000000000000, 1.000000000000000000 ) ) ;
#123947=DIRECTION ( 'NONE',  ( 0.000000000000000000, 0.000000000000000000, -1.000000000000000000 ) ) ;
#123948=AXIS2_PLACEMENT_3D ( 'NONE', #122911, #13577, #92144 ) ;
#123949=AXIS2_PLACEMENT_3D ( 'NONE', #108580, #88268, #78499 ) ;
#123950=AXIS2_PLACEMENT_3D ( 'NONE', #54927, #85030, #124972 ) ;
#123951=LINE ( 'NONE', #114144, #52791 ) ;
#123953=DIRECTION ( 'NONE',  ( 0.000000000000000000, 1.000000000000000000, 0.000000000000000000 ) ) ;
#123954=CARTESIAN_POINT ( 'NONE',  ( 6.699999999999930012, 2.500000000000000000, 4.330127018922196314 ) ) ;
#123955=VECTOR ( 'NONE', #10311, 1000.000000000000000 ) ;
#123956=DIRECTION ( 'NONE',  ( 0.000000000000000000, 1.000000000000000000, 0.000000000000000000 ) ) ;
#123957=ORIENTED_EDGE ( 'NONE', *, *, #101850, .F. ) ;
#123958=CONICAL_SURFACE ( 'NONE', #44554, 0.1000000000000002554, 0.003490658503988666988 ) ;
#123959=VERTEX_POINT ( 'NONE', #85145 ) ;
#123960=ORIENTED_EDGE ( 'NONE', *, *, #86057, .F. ) ;
#123961=ORIENTED_EDGE ( 'NONE', *, *, #13004, .T. ) ;
#123962=DIRECTION ( 'NONE',  ( 0.000000000000000000, 1.000000000000000000, 0.000000000000000000 ) ) ;
#123963=LINE ( 'NONE', #13368, #123095 ) ;
#123964=CARTESIAN_POINT ( 'NONE',  ( 3.349999999999945466, 12.50000000000000000, -6.560283801567339701 ) ) ;
#123965=ORIENTED_EDGE ( 'NONE', *, *, #94959, .F. ) ;
#123966=FACE_BOUND ( 'NONE', #73108, .T. ) ;
#123967=DIRECTION ( 'NONE',  ( -0.000000000000000000, 1.000000000000000000, -0.000000000000000000 ) ) ;
#123968=DIRECTION ( 'NONE',  ( 0.000000000000000000, 0.000000000000000000, -1.000000000000000000 ) ) ;
#123969=CARTESIAN_POINT ( 'NONE',  ( -4.550000000000022915, 12.50000000000000000, 6.495190528383297135 ) ) ;
#123970=DIRECTION ( 'NONE',  ( 0.000000000000000000, -0.000000000000000000, 1.000000000000000000 ) ) ;
#123971=DIRECTION ( 'NONE',  ( 0.000000000000000000, -0.000000000000000000, 1.000000000000000000 ) ) ;
#123973=PLANE ( 'NONE',  #64289 ) ;
#123974=DIRECTION ( 'NONE',  ( 0.000000000000000000, 0.000000000000000000, 1.000000000000000000 ) ) ;
#123975=AXIS2_PLACEMENT_3D ( 'NONE', #41934, #81832, #82504 ) ;
#123976=DIRECTION ( 'NONE',  ( -0.000000000000000000, -1.000000000000000000, -0.000000000000000000 ) ) ;
#123977=CARTESIAN_POINT ( 'NONE',  ( 7.699999999999923794, 12.50000000000000000, -3.918623584224389056 ) ) ;
#123978=ORIENTED_EDGE ( 'NONE', *, *, #92914, .T. ) ;
#123979=ADVANCED_FACE ( 'NONE', ( #75325 ), #115220, .T. ) ;
#123980=VECTOR ( 'NONE', #42981, 1000.000000000000000 ) ;
#123981=ORIENTED_EDGE ( 'NONE', *, *, #82485, .F. ) ;
#123982=EDGE_LOOP ( 'NONE', ( #6952, #76381, #36387, #10424 ) ) ;
#123983=EDGE_LOOP ( 'NONE', ( #77819, #55103, #43254, #45335 ) ) ;
#123984=AXIS2_PLACEMENT_3D ( 'NONE', #91608, #41240, #52327 ) ;
#123985=EDGE_LOOP ( 'NONE', ( #30007, #90853, #66213, #47094 ) ) ;
#123986=VECTOR ( 'NONE', #79733, 1000.000000000000000 ) ;
#123987=ORIENTED_EDGE ( 'NONE', *, *, #86649, .F. ) ;
#123988=CONICAL_SURFACE ( 'NONE', #29913, 0.1000000000000000472, 0.003490658503988666988 ) ;
#123989=DIRECTION ( 'NONE',  ( 0.000000000000000000, 1.000000000000000000, 0.000000000000000000 ) ) ;
#123990=ORIENTED_EDGE ( 'NONE', *, *, #118368, .T. ) ;
#123991=EDGE_LOOP ( 'NONE', ( #5449, #88188, #49039, #104477 ) ) ;
#123992=EDGE_CURVE ( 'NONE', #79185, #126997, #37662, .T. ) ;
#123993=VECTOR ( 'NONE', #108124, 1000.000000000000000 ) ;
#123994=VECTOR ( 'NONE', #5721, 1000.000000000000000 ) ;
#123995=VECTOR ( 'NONE', #22506, 1000.000000000000000 ) ;
#123996=CARTESIAN_POINT ( 'NONE',  ( 9.112263991918540640, -2.499999999999490630, 9.392448312006209221 ) ) ;
#123997=CARTESIAN_POINT ( 'NONE',  ( -11.69999999999999929, 2.500000000000000000, -4.430127018922199511 ) ) ;
#123998=DIRECTION ( 'NONE',  ( -4.274815082592931898E-19, -0.9999939076577903929, -0.003490651415223739937 ) ) ;
#123999=AXIS2_PLACEMENT_3D ( 'NONE', #98712, #100026, #10347 ) ;
#124000=DIRECTION ( 'NONE',  ( 0.000000000000000000, 0.000000000000000000, -1.000000000000000000 ) ) ;
#124001=VECTOR ( 'NONE', #80583, 1000.000000000000000 ) ;
#124002=EDGE_CURVE ( 'NONE', #907, #36869, #36713, .T. ) ;
#124003=ADVANCED_FACE ( 'NONE', ( #69368 ), #126371, .T. ) ;
#124004=ORIENTED_EDGE ( 'NONE', *, *, #119584, .F. ) ;
#124005=DIRECTION ( 'NONE',  ( 0.000000000000000000, 0.000000000000000000, 1.000000000000000000 ) ) ;
#124006=AXIS2_PLACEMENT_3D ( 'NONE', #79939, #90387, #89762 ) ;
#124007=ORIENTED_EDGE ( 'NONE', *, *, #126536, .F. ) ;
#124008=ORIENTED_EDGE ( 'NONE', *, *, #68212, .F. ) ;
#124009=PLANE ( 'NONE',  #7080 ) ;
#124010=ORIENTED_EDGE ( 'NONE', *, *, #115399, .T. ) ;
#124011=ADVANCED_FACE ( 'NONE', ( #99499 ), #47821, .T. ) ;
#124012=CARTESIAN_POINT ( 'NONE',  ( -6.450000000000019718, 12.50000000000000000, -6.083687093685488989 ) ) ;
#124013=ORIENTED_EDGE ( 'NONE', *, *, #93303, .T. ) ;
#124014=ADVANCED_FACE ( 'NONE', ( #46505 ), #96209, .T. ) ;
#124015=ORIENTED_EDGE ( 'NONE', *, *, #14023, .F. ) ;
#124016=AXIS2_PLACEMENT_3D ( 'NONE', #114748, #22537, #24447 ) ;
#124017=DIRECTION ( 'NONE',  ( 0.000000000000000000, 0.000000000000000000, -1.000000000000000000 ) ) ;
#124018=CARTESIAN_POINT ( 'NONE',  ( 3.349999999999945466, 2.500000000000000000, -2.165063509461101710 ) ) ;
#124019=DIRECTION ( 'NONE',  ( 0.000000000000000000, 0.000000000000000000, -1.000000000000000000 ) ) ;
#124020=DIRECTION ( 'NONE',  ( 0.000000000000000000, 0.000000000000000000, 1.000000000000000000 ) ) ;
#124021=DIRECTION ( 'NONE',  ( 0.000000000000000000, 0.000000000000000000, 1.000000000000000000 ) ) ;
#124022=CONICAL_SURFACE ( 'NONE', #107389, 0.1000000000000002554, 0.003490658503988666988 ) ;
#124023=EDGE_LOOP ( 'NONE', ( #119180, #91519 ) ) ;
#124024=DIRECTION ( 'NONE',  ( -4.274815082592931898E-19, -0.9999939076577903929, -0.003490651415223739937 ) ) ;
#124027=EDGE_LOOP ( 'NONE', ( #72195, #108243, #30559, #37535 ) ) ;
#124028=CARTESIAN_POINT ( 'NONE',  ( 17.50000000000000000, 2.499999999999999556, -2.666666666666662522 ) ) ;
#124029=EDGE_LOOP ( 'NONE', ( #18045, #106743 ) ) ;
#124031=EDGE_CURVE ( 'NONE', #46603, #26800, #38659, .T. ) ;
#124032=DIRECTION ( 'NONE',  ( -0.000000000000000000, -1.000000000000000000, -0.000000000000000000 ) ) ;
#124033=DIRECTION ( 'NONE',  ( 0.000000000000000000, 0.000000000000000000, -1.000000000000000000 ) ) ;
#124034=LINE ( 'NONE', #105030, #35490 ) ;
#124035=AXIS2_PLACEMENT_3D ( 'NONE', #62148, #97384, #27337 ) ;
#124036=ORIENTED_EDGE ( 'NONE', *, *, #35102, .T. ) ;
#124037=AXIS2_PLACEMENT_3D ( 'NONE', #95991, #64586, #12418 ) ;
#124038=CIRCLE ( 'NONE', #67589, 0.09999999999999999167 ) ;
#124039=EDGE_CURVE ( 'NONE', #103404, #36921, #121278, .T. ) ;
#124040=DIRECTION ( 'NONE',  ( -0.000000000000000000, 1.000000000000000000, -0.000000000000000000 ) ) ;
#124041=ORIENTED_EDGE ( 'NONE', *, *, #124956, .T. ) ;
#124042=ORIENTED_EDGE ( 'NONE', *, *, #37034, .T. ) ;
#124043=ORIENTED_EDGE ( 'NONE', *, *, #30251, .F. ) ;
#124044=DIRECTION ( 'NONE',  ( 0.000000000000000000, 0.000000000000000000, 1.000000000000000000 ) ) ;
#124045=DIRECTION ( 'NONE',  ( 0.000000000000000000, 0.000000000000000000, -1.000000000000000000 ) ) ;
#124047=AXIS2_PLACEMENT_3D ( 'NONE', #43680, #30147, #99530 ) ;
#124048=LINE ( 'NONE', #125972, #3174 ) ;
#124049=ADVANCED_FACE ( 'NONE', ( #108655 ), #112955, .T. ) ;
#124051=AXIS2_PLACEMENT_3D ( 'NONE', #50684, #88005, #68387 ) ;
#124052=CIRCLE ( 'NONE', #42506, 0.09999999999999982514 ) ;
#124053=DIRECTION ( 'NONE',  ( 0.000000000000000000, 0.000000000000000000, 1.000000000000000000 ) ) ;
#124054=ADVANCED_FACE ( 'NONE', ( #68731 ), #125474, .T. ) ;
#124055=VECTOR ( 'NONE', #127996, 1000.000000000000000 ) ;
#124056=EDGE_CURVE ( 'NONE', #97932, #73695, #89876, .T. ) ;
#124057=EDGE_CURVE ( 'NONE', #110043, #128895, #2141, .T. ) ;
#124058=EDGE_LOOP ( 'NONE', ( #42427, #97028 ) ) ;
#124059=CARTESIAN_POINT ( 'NONE',  ( 7.099999999999927702, 12.50000000000000000, -3.637306695894650055 ) ) ;
#124060=ORIENTED_EDGE ( 'NONE', *, *, #91887, .F. ) ;
#124061=EDGE_CURVE ( 'NONE', #14140, #65023, #66884, .T. ) ;
#124063=CARTESIAN_POINT ( 'NONE',  ( 7.899999999999924860, 12.50000000000000000, -3.572213422710612374 ) ) ;
#124064=CARTESIAN_POINT ( 'NONE',  ( -9.999999999999969802, 2.500000000000000000, -0.1000000000000022815 ) ) ;
#124065=VERTEX_POINT ( 'NONE', #106712 ) ;
#124066=ADVANCED_FACE ( 'NONE', ( #8507 ), #33460, .T. ) ;
#124067=EDGE_CURVE ( 'NONE', #37140, #36953, #58285, .T. ) ;
#124068=FACE_OUTER_BOUND ( 'NONE', #69182, .T. ) ;
#124069=DIRECTION ( 'NONE',  ( 0.000000000000000000, 0.000000000000000000, 1.000000000000000000 ) ) ;
#124070=VECTOR ( 'NONE', #6464, 1000.000000000000000 ) ;
#124071=CONICAL_SURFACE ( 'NONE', #67630, 0.1000000000000002554, 0.003490658503988666988 ) ;
#124072=VERTEX_POINT ( 'NONE', #7870 ) ;
#124073=LINE ( 'NONE', #12810, #90685 ) ;
#124074=CIRCLE ( 'NONE', #25879, 0.09999999999999982514 ) ;
#124075=CIRCLE ( 'NONE', #84371, 0.06509327318403745899 ) ;
#124076=EDGE_LOOP ( 'NONE', ( #69339, #114134, #92610, #125638 ) ) ;
#124077=AXIS2_PLACEMENT_3D ( 'NONE', #18191, #79072, #118334 ) ;
#124078=ORIENTED_EDGE ( 'NONE', *, *, #57255, .F. ) ;
#124079=CARTESIAN_POINT ( 'NONE',  ( -1.450000000000036371, 2.500000000000000000, 6.841600689897072485 ) ) ;
#124080=CIRCLE ( 'NONE', #11207, 0.1000000000000002554 ) ;
#124081=CONICAL_SURFACE ( 'NONE', #92695, 0.1000000000000002554, 0.003490658503988666988 ) ;
#124082=ORIENTED_EDGE ( 'NONE', *, *, #109678, .F. ) ;
#124083=CARTESIAN_POINT ( 'NONE',  ( -12.69999999999999041, 2.500000000000000000, 3.983716857408420964 ) ) ;
#124084=DIRECTION ( 'NONE',  ( 0.000000000000000000, 1.000000000000000000, 0.000000000000000000 ) ) ;
#124085=CARTESIAN_POINT ( 'NONE',  ( -9.150000000000009237, 2.500000000000000000, -7.188010851410848723 ) ) ;
#124086=VERTEX_POINT ( 'NONE', #28825 ) ;
#124087=CIRCLE ( 'NONE', #84378, 0.1000000000000002554 ) ;
#124088=CIRCLE ( 'NONE', #101107, 0.06509327318403745899 ) ;
#124089=CARTESIAN_POINT ( 'NONE',  ( 5.449999999999936229, 2.500000000000000000, -2.265063509461101798 ) ) ;
#124090=CARTESIAN_POINT ( 'NONE',  ( -11.25000000000000000, 12.50000000000000000, -2.792790559304612508 ) ) ;
#124092=CIRCLE ( 'NONE', #63464, 0.1000000000000002554 ) ;
#124093=CARTESIAN_POINT ( 'NONE',  ( -6.850000000000017408, 2.500000000000000000, -1.918653347947325782 ) ) ;
#124094=LINE ( 'NONE', #115543, #25834 ) ;
#124095=ORIENTED_EDGE ( 'NONE', *, *, #83944, .F. ) ;
#124097=EDGE_LOOP ( 'NONE', ( #27325, #126905 ) ) ;
#124098=DIRECTION ( 'NONE',  ( 0.000000000000000000, -0.000000000000000000, 1.000000000000000000 ) ) ;
#124099=DIRECTION ( 'NONE',  ( -4.274815082592931898E-19, -0.9999939076577903929, -0.003490651415223739937 ) ) ;
#124100=DIRECTION ( 'NONE',  ( 0.000000000000000000, 0.000000000000000000, -1.000000000000000000 ) ) ;
#124101=FACE_BOUND ( 'NONE', #18963, .T. ) ;
#124102=ORIENTED_EDGE ( 'NONE', *, *, #75003, .T. ) ;
#124104=DIRECTION ( 'NONE',  ( -4.274815082592931898E-19, -0.9999939076577903929, -0.003490651415223739937 ) ) ;
#124105=CARTESIAN_POINT ( 'NONE',  ( -10.40000000000000213, 2.500000000000000000, 4.922947341949748257 ) ) ;
#124106=AXIS2_PLACEMENT_3D ( 'NONE', #112678, #32202, #123140 ) ;
#124107=ADVANCED_FACE ( 'NONE', ( #77898 ), #118472, .T. ) ;
#124108=DIRECTION ( 'NONE',  ( -0.000000000000000000, -1.000000000000000000, -0.000000000000000000 ) ) ;
#124109=CARTESIAN_POINT ( 'NONE',  ( -7.100000000000018296, 2.500000000000000000, -2.385244779468109755E-15 ) ) ;
#124110=DIRECTION ( 'NONE',  ( -0.000000000000000000, -1.000000000000000000, -0.000000000000000000 ) ) ;
#124111=AXIS2_PLACEMENT_3D ( 'NONE', #69834, #60035, #99942 ) ;
#124112=AXIS2_PLACEMENT_3D ( 'NONE', #23034, #40765, #10606 ) ;
#124113=AXIS2_PLACEMENT_3D ( 'NONE', #18646, #57296, #97850 ) ;
#124114=FACE_OUTER_BOUND ( 'NONE', #54402, .T. ) ;
#124115=EDGE_LOOP ( 'NONE', ( #7197, #47925 ) ) ;
#124116=VERTEX_POINT ( 'NONE', #39313 ) ;
#124117=ORIENTED_EDGE ( 'NONE', *, *, #119183, .F. ) ;
#124118=ORIENTED_EDGE ( 'NONE', *, *, #120735, .T. ) ;
#124119=ORIENTED_EDGE ( 'NONE', *, *, #26222, .T. ) ;
#124120=CARTESIAN_POINT ( 'NONE',  ( 3.299999999999944755, 2.500000000000000000, -0.1000000000000023925 ) ) ;
#124121=CARTESIAN_POINT ( 'NONE',  ( -11.44999999999999929, 2.500000000000000000, -6.048780366869523029 ) ) ;
#124122=ORIENTED_EDGE ( 'NONE', *, *, #57550, .F. ) ;
#124123=FACE_BOUND ( 'NONE', #116117, .T. ) ;
#124124=CIRCLE ( 'NONE', #82382, 0.06509327318403745899 ) ;
#124125=CIRCLE ( 'NONE', #113672, 0.1000000000000002554 ) ;
#124126=CARTESIAN_POINT ( 'NONE',  ( 3.099999999999945022, 12.50000000000000000, -0.2813168883297409439 ) ) ;
#124127=VECTOR ( 'NONE', #103076, 1000.000000000000000 ) ;
#124128=CONICAL_SURFACE ( 'NONE', #78179, 0.1000000000000002554, 0.003490658503988666988 ) ;
#124129=CARTESIAN_POINT ( 'NONE',  ( 1.849999999999950129, 2.500000000000000000, -6.741600689897078169 ) ) ;
#124130=ORIENTED_EDGE ( 'NONE', *, *, #79815, .F. ) ;
#124131=CARTESIAN_POINT ( 'NONE',  ( 7.949999999999922018, 2.500000000000000000, -2.165063509461101710 ) ) ;
#124132=FACE_OUTER_BOUND ( 'NONE', #13329, .T. ) ;
#124133=DIRECTION ( 'NONE',  ( 0.000000000000000000, 1.000000000000000000, 0.000000000000000000 ) ) ;
#124134=CONICAL_SURFACE ( 'NONE', #96943, 0.1000000000000000472, 0.003490658503988666988 ) ;
#124135=ORIENTED_EDGE ( 'NONE', *, *, #113836, .F. ) ;
#124136=FACE_OUTER_BOUND ( 'NONE', #441, .T. ) ;
#124137=ORIENTED_EDGE ( 'NONE', *, *, #68874, .F. ) ;
#124138=CIRCLE ( 'NONE', #19595, 0.06509327318403745899 ) ;
#124140=VECTOR ( 'NONE', #61234, 1000.000000000000000 ) ;
#124141=ORIENTED_EDGE ( 'NONE', *, *, #5834, .T. ) ;
#124142=EDGE_LOOP ( 'NONE', ( #46258, #97296, #6295, #47618 ) ) ;
#124143=FACE_OUTER_BOUND ( 'NONE', #45991, .T. ) ;
#124144=DIRECTION ( 'NONE',  ( 0.000000000000000000, 0.000000000000000000, -1.000000000000000000 ) ) ;
#124145=LINE ( 'NONE', #102564, #67595 ) ;
#124146=CIRCLE ( 'NONE', #126307, 0.06509327318403745899 ) ;
#124147=ORIENTED_EDGE ( 'NONE', *, *, #118762, .F. ) ;
#124148=DIRECTION ( 'NONE',  ( -4.274815082592931898E-19, -0.9999939076577903929, -0.003490651415223739937 ) ) ;
#124149=VECTOR ( 'NONE', #94477, 1000.000000000000000 ) ;
#124150=ADVANCED_FACE ( 'NONE', ( #18978 ), #79516, .T. ) ;
#124152=DIRECTION ( 'NONE',  ( -4.274815082592931898E-19, -0.9999939076577903929, -0.003490651415223739937 ) ) ;
#124154=ORIENTED_EDGE ( 'NONE', *, *, #103221, .T. ) ;
#124155=ADVANCED_FACE ( 'NONE', ( #89028 ), #29464, .T. ) ;
#124156=DIRECTION ( 'NONE',  ( -0.000000000000000000, -1.000000000000000000, -0.000000000000000000 ) ) ;
#124157=EDGE_CURVE ( 'NONE', #68489, #99244, #77367, .T. ) ;
#124158=ORIENTED_EDGE ( 'NONE', *, *, #91696, .F. ) ;
#124160=ORIENTED_EDGE ( 'NONE', *, *, #41313, .T. ) ;
#124161=ORIENTED_EDGE ( 'NONE', *, *, #99975, .F. ) ;
#124162=DIRECTION ( 'NONE',  ( 0.000000000000000000, 0.000000000000000000, -1.000000000000000000 ) ) ;
#124163=DIRECTION ( 'NONE',  ( 0.000000000000000000, 0.000000000000000000, 1.000000000000000000 ) ) ;
#124164=EDGE_CURVE ( 'NONE', #62242, #49122, #81562, .T. ) ;
#124165=EDGE_CURVE ( 'NONE', #46262, #40507, #54366, .T. ) ;
#124166=AXIS2_PLACEMENT_3D ( 'NONE', #62709, #102609, #71220 ) ;
#124167=CARTESIAN_POINT ( 'NONE',  ( -5.600000000000023626, 2.500000000000000000, -4.576537180435977348 ) ) ;
#124168=ADVANCED_FACE ( 'NONE', ( #50384 ), #71977, .T. ) ;
#124169=LINE ( 'NONE', #54145, #13271 ) ;
#124170=EDGE_CURVE ( 'NONE', #515, #120902, #87807, .T. ) ;
#124171=DIRECTION ( 'NONE',  ( 0.000000000000000000, 0.000000000000000000, -1.000000000000000000 ) ) ;
#124172=EDGE_LOOP ( 'NONE', ( #93418, #7293, #50724, #1289 ) ) ;
#124173=VERTEX_POINT ( 'NONE', #70034 ) ;
#124174=CARTESIAN_POINT ( 'NONE',  ( 11.64999999999990798, 2.500000000000000000, -1.572243186433550211 ) ) ;
#124175=AXIS2_PLACEMENT_3D ( 'NONE', #123919, #64361, #44081 ) ;
#124176=AXIS2_PLACEMENT_3D ( 'NONE', #94581, #123401, #42952 ) ;
#124177=AXIS2_PLACEMENT_3D ( 'NONE', #28458, #109592, #126652 ) ;
#124178=CARTESIAN_POINT ( 'NONE',  ( 8.749999999999923617, 2.500000000000000000, -7.088010851410853519 ) ) ;
#124179=AXIS2_PLACEMENT_3D ( 'NONE', #105002, #74277, #85377 ) ;
#124180=FACE_OUTER_BOUND ( 'NONE', #77995, .T. ) ;
#124182=ORIENTED_EDGE ( 'NONE', *, *, #74992, .F. ) ;
#124183=VERTEX_POINT ( 'NONE', #42523 ) ;
#124184=PLANE ( 'NONE',  #72855 ) ;
#124185=EDGE_CURVE ( 'NONE', #12221, #2395, #64825, .T. ) ;
#124186=ORIENTED_EDGE ( 'NONE', *, *, #8047, .F. ) ;
#124187=CARTESIAN_POINT ( 'NONE',  ( 8.949999999999915801, 2.500000000000000000, 6.841600689897072485 ) ) ;
#124188=AXIS2_PLACEMENT_3D ( 'NONE', #28136, #88314, #97509 ) ;
#124189=CONICAL_SURFACE ( 'NONE', #107459, 0.09999999999999982514, 0.003490658503988666988 ) ;
#124190=VECTOR ( 'NONE', #128992, 1000.000000000000000 ) ;
#124191=DIRECTION ( 'NONE',  ( 0.000000000000000000, 0.000000000000000000, -1.000000000000000000 ) ) ;
#124192=VERTEX_POINT ( 'NONE', #20281 ) ;
#124193=FACE_OUTER_BOUND ( 'NONE', #17185, .T. ) ;
#124194=CARTESIAN_POINT ( 'NONE',  ( -7.300000000000016698, 2.500000000000000000, -0.3464101615137783474 ) ) ;
#124195=LINE ( 'NONE', #126121, #99041 ) ;
#124196=CARTESIAN_POINT ( 'NONE',  ( 7.099999999999928590, 2.500000000000000000, -4.330127018922201643 ) ) ;
#124197=VERTEX_POINT ( 'NONE', #52321 ) ;
#124198=DIRECTION ( 'NONE',  ( 0.000000000000000000, 1.000000000000000000, 0.000000000000000000 ) ) ;
#124199=CARTESIAN_POINT ( 'NONE',  ( 1.699999999999950218, 2.500000000000000000, 4.330127018922196314 ) ) ;
#124200=CONICAL_SURFACE ( 'NONE', #113445, 0.1000000000000002554, 0.003490658503988666988 ) ;
#124201=EDGE_LOOP ( 'NONE', ( #12452, #77442 ) ) ;
#124202=ORIENTED_EDGE ( 'NONE', *, *, #33783, .F. ) ;
#124203=EDGE_CURVE ( 'NONE', #44929, #114153, #9818, .T. ) ;
#124204=CARTESIAN_POINT ( 'NONE',  ( 3.749999999999942268, 12.50000000000000000, -5.737276932171712751 ) ) ;
#124205=CARTESIAN_POINT ( 'NONE',  ( 6.849999999999927702, 2.500000000000000000, 1.818653347947321475 ) ) ;
#124206=DIRECTION ( 'NONE',  ( 0.000000000000000000, 0.000000000000000000, 1.000000000000000000 ) ) ;
#124207=CIRCLE ( 'NONE', #99082, 0.06509327318403745899 ) ;
#124208=FACE_OUTER_BOUND ( 'NONE', #22228, .T. ) ;
#124209=DIRECTION ( 'NONE',  ( 0.000000000000000000, 1.000000000000000000, 0.000000000000000000 ) ) ;
#124210=DIRECTION ( 'NONE',  ( 0.000000000000000000, 0.000000000000000000, 1.000000000000000000 ) ) ;
#124211=CARTESIAN_POINT ( 'NONE',  ( 4.399999999999940847, 2.500000000000000000, -4.676537180435977881 ) ) ;
#124212=LINE ( 'NONE', #2485, #7286 ) ;
#124213=DIRECTION ( 'NONE',  ( -4.274815082592931898E-19, -0.9999939076577903929, -0.003490651415223739937 ) ) ;
#124214=CARTESIAN_POINT ( 'NONE',  ( -7.100000000000018296, 2.500000000000000000, -0.1000000000000023925 ) ) ;
#124215=EDGE_CURVE ( 'NONE', #38646, #6835, #64919, .T. ) ;
#124216=ADVANCED_FACE ( 'NONE', ( #41871 ), #31406, .T. ) ;
#124218=CARTESIAN_POINT ( 'NONE',  ( 8.149999999999920419, 2.500000000000000000, 6.248780366869521430 ) ) ;
#124219=VECTOR ( 'NONE', #60717, 1000.000000000000000 ) ;
#124220=ORIENTED_EDGE ( 'NONE', *, *, #113398, .T. ) ;
#124221=CIRCLE ( 'NONE', #63583, 0.06509327318403745899 ) ;
#124222=ORIENTED_EDGE ( 'NONE', *, *, #96394, .F. ) ;
#124223=ORIENTED_EDGE ( 'NONE', *, *, #97394, .F. ) ;
#124224=ADVANCED_FACE ( 'NONE', ( #101425 ), #6401, .T. ) ;
#124225=ORIENTED_EDGE ( 'NONE', *, *, #6816, .T. ) ;
#124226=ADVANCED_FACE ( 'NONE', ( #22233 ), #77446, .T. ) ;
#124227=DIRECTION ( 'NONE',  ( 0.000000000000000000, 0.000000000000000000, 1.000000000000000000 ) ) ;
#124228=CARTESIAN_POINT ( 'NONE',  ( 11.64999999999990443, 12.50000000000000000, -5.802370205355749988 ) ) ;
#124229=DIRECTION ( 'NONE',  ( 0.000000000000000000, 1.000000000000000000, 0.000000000000000000 ) ) ;
#124230=ADVANCED_FACE ( 'NONE', ( #11087 ), #100435, .T. ) ;
#124231=ORIENTED_EDGE ( 'NONE', *, *, #13676, .F. ) ;
#124232=EDGE_CURVE ( 'NONE', #45669, #92207, #2217, .T. ) ;
#124233=DIRECTION ( 'NONE',  ( -0.000000000000000000, 1.000000000000000000, -0.000000000000000000 ) ) ;
#124234=VECTOR ( 'NONE', #14596, 1000.000000000000000 ) ;
#124235=ADVANCED_FACE ( 'NONE', ( #41233 ), #4263, .T. ) ;
#124236=DIRECTION ( 'NONE',  ( 0.000000000000000000, 1.000000000000000000, 0.000000000000000000 ) ) ;
#124237=DIRECTION ( 'NONE',  ( 0.000000000000000000, 0.000000000000000000, -1.000000000000000000 ) ) ;
#124238=VERTEX_POINT ( 'NONE', #51689 ) ;
#124239=DIRECTION ( 'NONE',  ( 0.000000000000000000, -0.000000000000000000, 1.000000000000000000 ) ) ;
#124240=EDGE_CURVE ( 'NONE', #69133, #78664, #106682, .T. ) ;
#124241=DIRECTION ( 'NONE',  ( -0.000000000000000000, 1.000000000000000000, -0.000000000000000000 ) ) ;
#124242=ORIENTED_EDGE ( 'NONE', *, *, #94338, .F. ) ;
#124243=CIRCLE ( 'NONE', #101251, 0.1000000000000002554 ) ;
#124244=AXIS2_PLACEMENT_3D ( 'NONE', #36418, #114943, #94667 ) ;
#124245=ORIENTED_EDGE ( 'NONE', *, *, #90608, .F. ) ;
#124246=ORIENTED_EDGE ( 'NONE', *, *, #104320, .F. ) ;
#124247=VERTEX_POINT ( 'NONE', #55383 ) ;
#124249=CIRCLE ( 'NONE', #9311, 0.1000000000000002554 ) ;
#124250=CARTESIAN_POINT ( 'NONE',  ( -2.900000000000029221, 2.500000000000000000, -4.922947341949753586 ) ) ;
#124251=DIRECTION ( 'NONE',  ( 0.000000000000000000, 0.000000000000000000, -1.000000000000000000 ) ) ;
#124252=CIRCLE ( 'NONE', #115833, 0.09999999999999982514 ) ;
#124253=DIRECTION ( 'NONE',  ( -4.274815082592931898E-19, -0.9999939076577903929, -0.003490651415223739937 ) ) ;
#124254=VERTEX_POINT ( 'NONE', #85482 ) ;
#124255=FACE_OUTER_BOUND ( 'NONE', #67129, .T. ) ;
#124258=CARTESIAN_POINT ( 'NONE',  ( -7.050000000000013145, 2.500000000000000000, 6.395190528383296602 ) ) ;
#124259=FACE_OUTER_BOUND ( 'NONE', #72068, .T. ) ;
#124260=LINE ( 'NONE', #14285, #92355 ) ;
#124261=ORIENTED_EDGE ( 'NONE', *, *, #37368, .T. ) ;
#124262=AXIS2_PLACEMENT_3D ( 'NONE', #34055, #123691, #64788 ) ;
#124263=EDGE_LOOP ( 'NONE', ( #15063, #13701, #92606, #100438 ) ) ;
#124264=CONICAL_SURFACE ( 'NONE', #40663, 0.1000000000000002554, 0.003490658503988666988 ) ;
#124265=ORIENTED_EDGE ( 'NONE', *, *, #4401, .F. ) ;
#124266=CARTESIAN_POINT ( 'NONE',  ( -11.64999999999999680, 2.500000000000000000, -2.857883832488649745 ) ) ;
#124267=CARTESIAN_POINT ( 'NONE',  ( 7.099999999999926814, 12.50000000000000000, -0.6277270498435166823 ) ) ;
#124268=AXIS2_PLACEMENT_3D ( 'NONE', #374, #60625, #69780 ) ;
#124269=AXIS2_PLACEMENT_3D ( 'NONE', #16886, #127531, #128849 ) ;
#124270=LINE ( 'NONE', #5751, #77527 ) ;
#124271=FACE_BOUND ( 'NONE', #72943, .T. ) ;
#124272=DIRECTION ( 'NONE',  ( 0.000000000000000000, -0.9999939076577903929, 0.003490651415223739937 ) ) ;
#124273=CARTESIAN_POINT ( 'NONE',  ( 5.199999999999933564, 12.50000000000000000, 3.983716857408420076 ) ) ;
#124274=CARTESIAN_POINT ( 'NONE',  ( -11.44999999999999929, 2.500000000000000000, -6.148780366869522673 ) ) ;
#124275=AXIS2_PLACEMENT_3D ( 'NONE', #19540, #78486, #71216 ) ;
#124276=EDGE_CURVE ( 'NONE', #89750, #77424, #119296, .T. ) ;
#124277=AXIS2_PLACEMENT_3D ( 'NONE', #49794, #90320, #28857 ) ;
#124278=AXIS2_PLACEMENT_3D ( 'NONE', #1033, #13420, #91345 ) ;
#124280=CARTESIAN_POINT ( 'NONE',  ( -14.99999999999998224, 2.500000000000000000, -0.6928203230275519209 ) ) ;
#124281=DIRECTION ( 'NONE',  ( -0.000000000000000000, 1.000000000000000000, -0.000000000000000000 ) ) ;
#124282=EDGE_LOOP ( 'NONE', ( #74898, #18781 ) ) ;
#124283=VECTOR ( 'NONE', #92824, 1000.000000000000000 ) ;
#124284=CIRCLE ( 'NONE', #95042, 0.06509327318403745899 ) ;
#124285=DIRECTION ( 'NONE',  ( 0.000000000000000000, 0.000000000000000000, 1.000000000000000000 ) ) ;
#124286=ORIENTED_EDGE ( 'NONE', *, *, #118860, .F. ) ;
#124287=VERTEX_POINT ( 'NONE', #43168 ) ;
#124288=ORIENTED_EDGE ( 'NONE', *, *, #82710, .F. ) ;
#124289=VERTEX_POINT ( 'NONE', #3229 ) ;
#124290=AXIS2_PLACEMENT_3D ( 'NONE', #86195, #107793, #16801 ) ;
#124291=ADVANCED_FACE ( 'NONE', ( #37037 ), #127355, .T. ) ;
#124292=PLANE ( 'NONE',  #121717 ) ;
#124293=FACE_BOUND ( 'NONE', #45480, .T. ) ;
#124294=DIRECTION ( 'NONE',  ( 0.000000000000000000, 1.000000000000000000, 0.000000000000000000 ) ) ;
#124295=ORIENTED_EDGE ( 'NONE', *, *, #49592, .F. ) ;
#124296=DIRECTION ( 'NONE',  ( 0.000000000000000000, 0.000000000000000000, 1.000000000000000000 ) ) ;
#124297=CARTESIAN_POINT ( 'NONE',  ( -8.550000000000014921, 12.50000000000000000, -6.148780366869520897 ) ) ;
#124298=AXIS2_PLACEMENT_3D ( 'NONE', #23766, #6648, #34243 ) ;
#124299=ORIENTED_EDGE ( 'NONE', *, *, #35094, .T. ) ;
#124300=DIRECTION ( 'NONE',  ( 0.000000000000000000, 0.000000000000000000, -1.000000000000000000 ) ) ;
#124301=CARTESIAN_POINT ( 'NONE',  ( -2.100000000000033396, 12.50000000000000000, -5.022947341949754119 ) ) ;
#124302=VERTEX_POINT ( 'NONE', #87401 ) ;
#124303=PLANE ( 'NONE',  #65282 ) ;
#124304=DIRECTION ( 'NONE',  ( 0.000000000000000000, 0.000000000000000000, 1.000000000000000000 ) ) ;
#124305=AXIS2_PLACEMENT_3D ( 'NONE', #80206, #97891, #78926 ) ;
#124306=CIRCLE ( 'NONE', #88709, 0.06509327318403745899 ) ;
#124307=VERTEX_POINT ( 'NONE', #76955 ) ;
#124308=EDGE_CURVE ( 'NONE', #92862, #123556, #92107, .T. ) ;
#124309=FACE_OUTER_BOUND ( 'NONE', #36506, .T. ) ;
#124310=FACE_OUTER_BOUND ( 'NONE', #24652, .T. ) ;
#124311=CARTESIAN_POINT ( 'NONE',  ( 12.09999999999990550, 2.500000000000000000, -4.330127018922201643 ) ) ;
#124312=EDGE_LOOP ( 'NONE', ( #68537, #100038 ) ) ;
#124313=ORIENTED_EDGE ( 'NONE', *, *, #12632, .T. ) ;
#124314=DIRECTION ( 'NONE',  ( 0.000000000000000000, 1.000000000000000000, 0.000000000000000000 ) ) ;
#124315=EDGE_CURVE ( 'NONE', #126002, #96634, #105109, .T. ) ;
#124316=ORIENTED_EDGE ( 'NONE', *, *, #18494, .T. ) ;
#124317=DIRECTION ( 'NONE',  ( 0.000000000000000000, -0.9999939076577903929, 0.003490651415223739937 ) ) ;
#124318=DIRECTION ( 'NONE',  ( 0.000000000000000000, 1.000000000000000000, 0.000000000000000000 ) ) ;
#124319=AXIS2_PLACEMENT_3D ( 'NONE', #97046, #97683, #47307 ) ;
#124320=ORIENTED_EDGE ( 'NONE', *, *, #69128, .T. ) ;
#124321=CIRCLE ( 'NONE', #109948, 0.06509327318403745899 ) ;
#124322=FACE_OUTER_BOUND ( 'NONE', #34608, .T. ) ;
#124323=DIRECTION ( 'NONE',  ( -0.000000000000000000, 1.000000000000000000, -0.000000000000000000 ) ) ;
#124324=CARTESIAN_POINT ( 'NONE',  ( 3.549999999999943867, 2.500000000000000000, -1.718653347947326049 ) ) ;
#124326=EDGE_CURVE ( 'NONE', #97364, #60150, #125555, .T. ) ;
#124327=DIRECTION ( 'NONE',  ( -0.000000000000000000, -1.000000000000000000, -0.000000000000000000 ) ) ;
#124328=EDGE_CURVE ( 'NONE', #21032, #84876, #56008, .T. ) ;
#124329=EDGE_CURVE ( 'NONE', #66137, #41959, #110887, .T. ) ;
#124330=EDGE_CURVE ( 'NONE', #80079, #48784, #10536, .T. ) ;
#124331=FACE_OUTER_BOUND ( 'NONE', #2398, .T. ) ;
#124332=VERTEX_POINT ( 'NONE', #114928 ) ;
#124333=VERTEX_POINT ( 'NONE', #65174 ) ;
#124334=DIRECTION ( 'NONE',  ( 0.000000000000000000, 0.000000000000000000, 1.000000000000000000 ) ) ;
#124335=CIRCLE ( 'NONE', #105558, 0.1000000000000000472 ) ;
#124336=CARTESIAN_POINT ( 'NONE',  ( 1.849999999999949019, 12.50000000000000000, 6.841600689897072485 ) ) ;
#124337=FACE_OUTER_BOUND ( 'NONE', #23137, .T. ) ;
#124338=ORIENTED_EDGE ( 'NONE', *, *, #20285, .T. ) ;
#124339=ORIENTED_EDGE ( 'NONE', *, *, #35118, .T. ) ;
#124340=ORIENTED_EDGE ( 'NONE', *, *, #56022, .T. ) ;
#124341=CIRCLE ( 'NONE', #1003, 0.09999999999999982514 ) ;
#124342=EDGE_CURVE ( 'NONE', #84404, #44343, #127620, .T. ) ;
#124343=DIRECTION ( 'NONE',  ( 0.000000000000000000, 1.000000000000000000, 0.000000000000000000 ) ) ;
#124344=AXIS2_PLACEMENT_3D ( 'NONE', #91273, #1590, #11421 ) ;
#124345=EDGE_CURVE ( 'NONE', #82981, #72411, #71183, .T. ) ;
#124347=ADVANCED_FACE ( 'NONE', ( #86762 ), #16862, .T. ) ;
#124348=CARTESIAN_POINT ( 'NONE',  ( 12.89999999999990088, 12.50000000000000000, 4.330127018922196314 ) ) ;
#124350=DIRECTION ( 'NONE',  ( 0.000000000000000000, 0.000000000000000000, 1.000000000000000000 ) ) ;
#124351=CARTESIAN_POINT ( 'NONE',  ( 2.099999999999949463, 12.50000000000000000, -3.637306695894650055 ) ) ;
#124352=CARTESIAN_POINT ( 'NONE',  ( 7.699999999999923794, 2.500000000000000000, 4.676537180435972552 ) ) ;
#124353=CARTESIAN_POINT ( 'NONE',  ( 10.84999999999991260, 12.50000000000000000, 6.495190528383297135 ) ) ;
#124354=DIRECTION ( 'NONE',  ( 0.000000000000000000, 0.000000000000000000, -1.000000000000000000 ) ) ;
#124355=CARTESIAN_POINT ( 'NONE',  ( -5.400000000000019895, 12.50000000000000000, -2.276824562219559311E-15 ) ) ;
#124356=EDGE_LOOP ( 'NONE', ( #95015, #78617, #72416, #108212 ) ) ;
#124357=VECTOR ( 'NONE', #27434, 1000.000000000000000 ) ;
#124358=CIRCLE ( 'NONE', #44939, 0.09999999999999982514 ) ;
#124359=CARTESIAN_POINT ( 'NONE',  ( 10.44999999999991047, 12.50000000000000000, -6.560283801567339701 ) ) ;
#124360=CIRCLE ( 'NONE', #113899, 0.06509327318403745899 ) ;
#124361=AXIS2_PLACEMENT_3D ( 'NONE', #91805, #72818, #29824 ) ;
#124362=VERTEX_POINT ( 'NONE', #5611 ) ;
#124364=EDGE_LOOP ( 'NONE', ( #29406, #29813, #23437, #42230 ) ) ;
#124365=CARTESIAN_POINT ( 'NONE',  ( 6.449999999999930012, 2.500000000000000000, 1.818653347947321475 ) ) ;
#124366=DIRECTION ( 'NONE',  ( 0.000000000000000000, 0.000000000000000000, 1.000000000000000000 ) ) ;
#124368=AXIS2_PLACEMENT_3D ( 'NONE', #91193, #111467, #38408 ) ;
#124369=CARTESIAN_POINT ( 'NONE',  ( -2.950000000000033484, 2.500000000000000000, -6.495190528383302464 ) ) ;
#124370=AXIS2_PLACEMENT_3D ( 'NONE', #36948, #127900, #76869 ) ;
#124371=CARTESIAN_POINT ( 'NONE',  ( 8.099999999999923261, 2.500000000000000000, 3.883716857408420431 ) ) ;
#124372=FACE_OUTER_BOUND ( 'NONE', #53060, .T. ) ;
#124373=DIRECTION ( 'NONE',  ( 0.000000000000000000, 1.000000000000000000, 0.000000000000000000 ) ) ;
#124374=ORIENTED_EDGE ( 'NONE', *, *, #33067, .T. ) ;
#124375=DIRECTION ( 'NONE',  ( 0.000000000000000000, 0.000000000000000000, -1.000000000000000000 ) ) ;
#124376=AXIS2_PLACEMENT_3D ( 'NONE', #16816, #68522, #85588 ) ;
#124377=DIRECTION ( 'NONE',  ( 0.000000000000000000, 0.000000000000000000, 1.000000000000000000 ) ) ;
#124378=AXIS2_PLACEMENT_3D ( 'NONE', #127432, #59353, #66557 ) ;
#124379=ORIENTED_EDGE ( 'NONE', *, *, #64884, .F. ) ;
#124380=CIRCLE ( 'NONE', #82716, 0.06509327318403741736 ) ;
#124381=ORIENTED_EDGE ( 'NONE', *, *, #89241, .T. ) ;
#124383=CIRCLE ( 'NONE', #76357, 0.06509327318403745899 ) ;
#124384=ADVANCED_FACE ( 'NONE', ( #52969 ), #104627, .T. ) ;
#124385=VERTEX_POINT ( 'NONE', #25925 ) ;
#124386=DIRECTION ( 'NONE',  ( 0.000000000000000000, 0.000000000000000000, -1.000000000000000000 ) ) ;
#124387=FACE_OUTER_BOUND ( 'NONE', #126528, .T. ) ;
#124388=ADVANCED_FACE ( 'NONE', ( #75648 ), #69126, .T. ) ;
#124389=CARTESIAN_POINT ( 'NONE',  ( -1.250000000000001554, 12.50000000000000000, 6.560283801567334372 ) ) ;
#124390=CARTESIAN_POINT ( 'NONE',  ( -4.350000000000023626, 2.500000000000000000, 2.611473670974873151 ) ) ;
#124391=ADVANCED_FACE ( 'NONE', ( #67095 ), #102570, .T. ) ;
#124392=CARTESIAN_POINT ( 'NONE',  ( 10.44999999999991402, 2.500000000000000000, 6.495190528383297135 ) ) ;
#124393=ORIENTED_EDGE ( 'NONE', *, *, #129595, .F. ) ;
#124394=DIRECTION ( 'NONE',  ( 0.000000000000000000, 0.000000000000000000, 1.000000000000000000 ) ) ;
#124395=CARTESIAN_POINT ( 'NONE',  ( 7.099999999999928590, 2.500000000000000000, 3.537306695894645081 ) ) ;
#124396=CIRCLE ( 'NONE', #126457, 0.06509327318403745899 ) ;
#124397=EDGE_CURVE ( 'NONE', #98726, #85814, #46145, .T. ) ;
#124398=CARTESIAN_POINT ( 'NONE',  ( 6.449999999999931788, 2.500000000000000000, -6.048780366869526581 ) ) ;
#124399=ORIENTED_EDGE ( 'NONE', *, *, #48750, .F. ) ;
#124400=ORIENTED_EDGE ( 'NONE', *, *, #46942, .T. ) ;
#124401=EDGE_LOOP ( 'NONE', ( #119089, #97579 ) ) ;
#124402=DIRECTION ( 'NONE',  ( 0.000000000000000000, -0.9999939076577903929, 0.003490651415223739937 ) ) ;
#124403=CIRCLE ( 'NONE', #38751, 0.06509327318403745899 ) ;
#124404=DIRECTION ( 'NONE',  ( -4.274815082592931898E-19, -0.9999939076577903929, -0.003490651415223739937 ) ) ;
#124405=DIRECTION ( 'NONE',  ( 0.000000000000000000, 0.000000000000000000, 1.000000000000000000 ) ) ;
#124406=ORIENTED_EDGE ( 'NONE', *, *, #72327, .F. ) ;
#124407=DIRECTION ( 'NONE',  ( 0.000000000000000000, -0.9999939076577903929, 0.003490651415223739937 ) ) ;
#124408=CARTESIAN_POINT ( 'NONE',  ( 8.349999999999923261, 2.500000000000000000, -5.802370205355749988 ) ) ;
#124409=CARTESIAN_POINT ( 'NONE',  ( 13.54999999999989768, 2.500000000000000000, -2.611473670974877592 ) ) ;
#124410=FACE_OUTER_BOUND ( 'NONE', #123394, .T. ) ;
#124412=DIRECTION ( 'NONE',  ( 0.000000000000000000, 0.000000000000000000, 1.000000000000000000 ) ) ;
#124413=CONICAL_SURFACE ( 'NONE', #57518, 0.1000000000000002554, 0.003490658503988666988 ) ;
#124414=ORIENTED_EDGE ( 'NONE', *, *, #122875, .F. ) ;
#124415=DIRECTION ( 'NONE',  ( 0.000000000000000000, 0.000000000000000000, -1.000000000000000000 ) ) ;
#124416=CONICAL_SURFACE ( 'NONE', #122280, 0.09999999999999982514, 0.003490658503988666988 ) ;
#124417=ORIENTED_EDGE ( 'NONE', *, *, #110304, .T. ) ;
#124418=ORIENTED_EDGE ( 'NONE', *, *, #107530, .F. ) ;
#124419=DIRECTION ( 'NONE',  ( 0.000000000000000000, 0.000000000000000000, 1.000000000000000000 ) ) ;
#124420=DIRECTION ( 'NONE',  ( -0.000000000000000000, -1.000000000000000000, -0.000000000000000000 ) ) ;
#124421=CARTESIAN_POINT ( 'NONE',  ( 10.84999999999991260, 2.500000000000000000, -1.472243186433550122 ) ) ;
#124422=DIRECTION ( 'NONE',  ( 0.000000000000000000, 0.000000000000000000, -1.000000000000000000 ) ) ;
#124423=CARTESIAN_POINT ( 'NONE',  ( -11.24999999999996447, 2.500000000000000000, -2.165063509461097713 ) ) ;
#124424=ORIENTED_EDGE ( 'NONE', *, *, #38194, .F. ) ;
#124425=AXIS2_PLACEMENT_3D ( 'NONE', #25920, #126700, #75019 ) ;
#124426=EDGE_CURVE ( 'NONE', #120893, #36089, #23157, .T. ) ;
#124427=ORIENTED_EDGE ( 'NONE', *, *, #73835, .F. ) ;
#124428=DIRECTION ( 'NONE',  ( 0.000000000000000000, 0.000000000000000000, -1.000000000000000000 ) ) ;
#124429=DIRECTION ( 'NONE',  ( -0.000000000000000000, 1.000000000000000000, -0.000000000000000000 ) ) ;
#124430=DIRECTION ( 'NONE',  ( 0.000000000000000000, 0.000000000000000000, 1.000000000000000000 ) ) ;
#124431=DIRECTION ( 'NONE',  ( -0.000000000000000000, -1.000000000000000000, -0.000000000000000000 ) ) ;
#124432=EDGE_LOOP ( 'NONE', ( #52871, #116690, #17630, #38906 ) ) ;
#124433=CARTESIAN_POINT ( 'NONE',  ( -0.4000000000000331624, 12.50000000000000000, 0.06509327318403743123 ) ) ;
#124434=DIRECTION ( 'NONE',  ( -4.274815082592931898E-19, -0.9999939076577903929, -0.003490651415223739937 ) ) ;
#124435=ORIENTED_EDGE ( 'NONE', *, *, #85496, .F. ) ;
#124436=DIRECTION ( 'NONE',  ( -0.000000000000000000, 1.000000000000000000, -0.000000000000000000 ) ) ;
#124437=EDGE_CURVE ( 'NONE', #67445, #126716, #50715, .T. ) ;
#124438=AXIS2_PLACEMENT_3D ( 'NONE', #92965, #66061, #43872 ) ;
#124439=EDGE_LOOP ( 'NONE', ( #87982, #44022 ) ) ;
#124440=FACE_BOUND ( 'NONE', #6997, .T. ) ;
#124441=PLANE ( 'NONE',  #116163 ) ;
#124442=ORIENTED_EDGE ( 'NONE', *, *, #68950, .T. ) ;
#124443=CARTESIAN_POINT ( 'NONE',  ( 12.49999999999993960, 12.50000000000000000, 4.265033745738159077 ) ) ;
#124444=CARTESIAN_POINT ( 'NONE',  ( 1.849999999999948130, 2.500000000000000000, 6.048780366869520364 ) ) ;
#124445=VECTOR ( 'NONE', #89286, 1000.000000000000000 ) ;
#124446=AXIS2_PLACEMENT_3D ( 'NONE', #98883, #10495, #30165 ) ;
#124447=ORIENTED_EDGE ( 'NONE', *, *, #48952, .F. ) ;
#124448=ORIENTED_EDGE ( 'NONE', *, *, #120851, .F. ) ;
#124450=CARTESIAN_POINT ( 'NONE',  ( 12.69999999999990159, 12.50000000000000000, -3.918623584224389056 ) ) ;
#124451=CARTESIAN_POINT ( 'NONE',  ( 3.949999999999942446, 12.50000000000000000, -2.576566944158915184 ) ) ;
#124452=CIRCLE ( 'NONE', #22065, 0.1000000000000002554 ) ;
#124453=AXIS2_PLACEMENT_3D ( 'NONE', #77771, #89542, #129502 ) ;
#124454=AXIS2_PLACEMENT_3D ( 'NONE', #45332, #84601, #83935 ) ;
#124455=DIRECTION ( 'NONE',  ( 0.000000000000000000, 0.000000000000000000, 1.000000000000000000 ) ) ;
#124456=DIRECTION ( 'NONE',  ( -0.000000000000000000, 1.000000000000000000, -0.000000000000000000 ) ) ;
#124457=AXIS2_PLACEMENT_3D ( 'NONE', #32502, #72408, #33133 ) ;
#124458=DIRECTION ( 'NONE',  ( 0.000000000000000000, 0.000000000000000000, -1.000000000000000000 ) ) ;
#124459=FACE_OUTER_BOUND ( 'NONE', #115221, .T. ) ;
#124460=CONICAL_SURFACE ( 'NONE', #11585, 0.09999999999999982514, 0.003490658503988666988 ) ;
#124461=ORIENTED_EDGE ( 'NONE', *, *, #64475, .F. ) ;
#124463=EDGE_CURVE ( 'NONE', #112979, #43211, #96310, .T. ) ;
#124464=ORIENTED_EDGE ( 'NONE', *, *, #107376, .F. ) ;
#124465=DIRECTION ( 'NONE',  ( -0.000000000000000000, -1.000000000000000000, -0.000000000000000000 ) ) ;
#124467=DIRECTION ( 'NONE',  ( -0.000000000000000000, 1.000000000000000000, -0.000000000000000000 ) ) ;
#124468=AXIS2_PLACEMENT_3D ( 'NONE', #25519, #104100, #14413 ) ;
#124469=DIRECTION ( 'NONE',  ( 0.000000000000000000, -0.000000000000000000, 1.000000000000000000 ) ) ;
#124470=VERTEX_POINT ( 'NONE', #38332 ) ;
#124471=VERTEX_POINT ( 'NONE', #59918 ) ;
#124472=DIRECTION ( 'NONE',  ( 0.000000000000000000, 0.000000000000000000, 1.000000000000000000 ) ) ;
#124473=VERTEX_POINT ( 'NONE', #39639 ) ;
#124474=LINE ( 'NONE', #34824, #30421 ) ;
#124476=VERTEX_POINT ( 'NONE', #129304 ) ;
#124477=DIRECTION ( 'NONE',  ( 0.000000000000000000, -0.000000000000000000, 1.000000000000000000 ) ) ;
#124478=EDGE_CURVE ( 'NONE', #117938, #107, #301, .T. ) ;
#124479=DIRECTION ( 'NONE',  ( 0.000000000000000000, -0.9999939076577903929, 0.003490651415223739937 ) ) ;
#124480=CARTESIAN_POINT ( 'NONE',  ( 7.899999999999924860, 2.500000000000000000, -4.922947341949753586 ) ) ;
#124481=DIRECTION ( 'NONE',  ( 0.000000000000000000, 0.000000000000000000, 1.000000000000000000 ) ) ;
#124482=CARTESIAN_POINT ( 'NONE',  ( -10.00000000000000533, 12.50000000000000000, -5.022947341949749678 ) ) ;
#124483=CARTESIAN_POINT ( 'NONE',  ( 10.84999999999990905, 2.500000000000000000, 2.265063509461097357 ) ) ;
#124484=EDGE_CURVE ( 'NONE', #93441, #7770, #33636, .T. ) ;
#124485=EDGE_CURVE ( 'NONE', #11640, #96489, #69712, .T. ) ;
#124486=FACE_OUTER_BOUND ( 'NONE', #9904, .T. ) ;
#124487=CARTESIAN_POINT ( 'NONE',  ( 14.19999999999989626, 2.500000000000000000, -2.276824562219559311E-15 ) ) ;
#124488=ADVANCED_FACE ( 'NONE', ( #18020 ), #48795, .T. ) ;
#124489=ADVANCED_FACE ( 'NONE', ( #100460 ), #10612, .T. ) ;
#124490=VECTOR ( 'NONE', #32242, 1000.000000000000000 ) ;
#124491=CARTESIAN_POINT ( 'NONE',  ( -3.300000000000027800, 12.50000000000000000, -2.276824562219559311E-15 ) ) ;
#124492=ORIENTED_EDGE ( 'NONE', *, *, #21384, .T. ) ;
#124493=ORIENTED_EDGE ( 'NONE', *, *, #26549, .F. ) ;
#124494=VERTEX_POINT ( 'NONE', #68413 ) ;
#124495=DIRECTION ( 'NONE',  ( 0.000000000000000000, 0.000000000000000000, -1.000000000000000000 ) ) ;
#124496=VERTEX_POINT ( 'NONE', #78908 ) ;
#124497=EDGE_CURVE ( 'NONE', #70390, #122264, #4349, .T. ) ;
#124498=CARTESIAN_POINT ( 'NONE',  ( 9.149999999999920419, 2.500000000000000000, -7.188010851410854052 ) ) ;
#124499=EDGE_CURVE ( 'NONE', #35145, #18946, #104714, .T. ) ;
#124500=ORIENTED_EDGE ( 'NONE', *, *, #17602, .T. ) ;
#124501=EDGE_LOOP ( 'NONE', ( #95761, #121588, #33754, #67832 ) ) ;
#124502=AXIS2_PLACEMENT_3D ( 'NONE', #43348, #53789, #93722 ) ;
#124503=ORIENTED_EDGE ( 'NONE', *, *, #103114, .T. ) ;
#124504=EDGE_CURVE ( 'NONE', #127509, #104821, #37830, .T. ) ;
#124505=CARTESIAN_POINT ( 'NONE',  ( 5.599999999999933031, 12.50000000000000000, 0.3464101615137735735 ) ) ;
#124506=AXIS2_PLACEMENT_3D ( 'NONE', #29657, #127850, #97743 ) ;
#124507=CONICAL_SURFACE ( 'NONE', #13665, 0.1000000000000000472, 0.003490658503988666988 ) ;
#124508=EDGE_CURVE ( 'NONE', #102844, #11437, #52489, .T. ) ;
#124509=EDGE_CURVE ( 'NONE', #32011, #26682, #115166, .T. ) ;
#124510=DIRECTION ( 'NONE',  ( -0.000000000000000000, 1.000000000000000000, -0.000000000000000000 ) ) ;
#124511=DIRECTION ( 'NONE',  ( 0.000000000000000000, 1.000000000000000000, 0.000000000000000000 ) ) ;
#124512=LINE ( 'NONE', #56390, #112843 ) ;
#124513=DIRECTION ( 'NONE',  ( -4.274815082592931898E-19, -0.9999939076577903929, -0.003490651415223739937 ) ) ;
#124514=ORIENTED_EDGE ( 'NONE', *, *, #9392, .T. ) ;
#124515=EDGE_CURVE ( 'NONE', #39039, #36386, #48145, .T. ) ;
#124516=LINE ( 'NONE', #36129, #30918 ) ;
#124517=ORIENTED_EDGE ( 'NONE', *, *, #51846, .F. ) ;
#124518=VERTEX_POINT ( 'NONE', #88030 ) ;
#124519=ORIENTED_EDGE ( 'NONE', *, *, #38638, .T. ) ;
#124520=AXIS2_PLACEMENT_3D ( 'NONE', #48976, #117026, #19490 ) ;
#124521=DIRECTION ( 'NONE',  ( 0.000000000000000000, -0.9999939076577903929, 0.003490651415223739937 ) ) ;
#124522=ORIENTED_EDGE ( 'NONE', *, *, #45747, .F. ) ;
#124524=VERTEX_POINT ( 'NONE', #127987 ) ;
#124526=CARTESIAN_POINT ( 'NONE',  ( -12.89999999999999147, 2.500000000000000000, -5.122947341949751987 ) ) ;
#124527=VECTOR ( 'NONE', #52009, 1000.000000000000000 ) ;
#124528=CARTESIAN_POINT ( 'NONE',  ( 10.39999999999991154, 12.50000000000000000, -3.572213422710612374 ) ) ;
#124529=AXIS2_PLACEMENT_3D ( 'NONE', #49961, #116727, #17215 ) ;
#124530=DIRECTION ( 'NONE',  ( 0.000000000000000000, 1.000000000000000000, 0.000000000000000000 ) ) ;
#124531=DIRECTION ( 'NONE',  ( -0.000000000000000000, -1.000000000000000000, -0.000000000000000000 ) ) ;
#124532=CARTESIAN_POINT ( 'NONE',  ( -10.65000000000000391, 12.50000000000000000, -1.753560074763284682 ) ) ;
#124533=EDGE_LOOP ( 'NONE', ( #17697, #44662, #84730, #80981 ) ) ;
#124534=DIRECTION ( 'NONE',  ( -4.274815082592931898E-19, -0.9999939076577903929, -0.003490651415223739937 ) ) ;
#124535=ORIENTED_EDGE ( 'NONE', *, *, #64225, .F. ) ;
#124536=CARTESIAN_POINT ( 'NONE',  ( -0.8500000000000382805, 12.50000000000000000, -1.537336459617587581 ) ) ;
#124537=ORIENTED_EDGE ( 'NONE', *, *, #54147, .F. ) ;
#124538=CARTESIAN_POINT ( 'NONE',  ( -9.400000000000007461, 2.500000000000000000, 4.083716857408420609 ) ) ;
#124539=VERTEX_POINT ( 'NONE', #29161 ) ;
#124540=EDGE_LOOP ( 'NONE', ( #126632, #106544, #16552, #126501 ) ) ;
#124541=DIRECTION ( 'NONE',  ( 0.000000000000000000, 1.000000000000000000, 0.000000000000000000 ) ) ;
#124542=DIRECTION ( 'NONE',  ( -0.000000000000000000, -1.000000000000000000, -0.000000000000000000 ) ) ;
#124543=EDGE_CURVE ( 'NONE', #122392, #94085, #6489, .T. ) ;
#124545=AXIS2_PLACEMENT_3D ( 'NONE', #15204, #14573, #25053 ) ;
#124546=DIRECTION ( 'NONE',  ( 0.000000000000000000, 0.000000000000000000, -1.000000000000000000 ) ) ;
#124547=ADVANCED_FACE ( 'NONE', ( #99180 ), #49449, .T. ) ;
#124548=ORIENTED_EDGE ( 'NONE', *, *, #94666, .F. ) ;
#124549=DIRECTION ( 'NONE',  ( -0.000000000000000000, -1.000000000000000000, -0.000000000000000000 ) ) ;
#124550=EDGE_LOOP ( 'NONE', ( #96555, #73309, #7709, #95129 ) ) ;
#124551=CARTESIAN_POINT ( 'NONE',  ( 1.449999999999951772, 12.50000000000000000, -6.148780366869526226 ) ) ;
#124553=CARTESIAN_POINT ( 'NONE',  ( 8.949999999999919353, 12.50000000000000000, -6.148780366869526226 ) ) ;
#124554=CARTESIAN_POINT ( 'NONE',  ( -11.64999999999999858, 12.50000000000000000, -1.472243186433546125 ) ) ;
#124555=ADVANCED_FACE ( 'NONE', ( #42190 ), #19034, .T. ) ;
#124556=CARTESIAN_POINT ( 'NONE',  ( 7.499999999999961808, 12.50000000000000000, -4.265033745738164406 ) ) ;
#124557=EDGE_LOOP ( 'NONE', ( #83218, #120019 ) ) ;
#124558=VERTEX_POINT ( 'NONE', #101755 ) ;
#124559=AXIS2_PLACEMENT_3D ( 'NONE', #20572, #18628, #78864 ) ;
#124560=EDGE_LOOP ( 'NONE', ( #109489, #41462 ) ) ;
#124561=CONICAL_SURFACE ( 'NONE', #116135, 0.09999999999999982514, 0.003490658503988666988 ) ;
#124562=LINE ( 'NONE', #83352, #113391 ) ;
#124563=CARTESIAN_POINT ( 'NONE',  ( 8.749999999999957367, 2.500000000000000000, -6.495190528383302464 ) ) ;
#124564=CIRCLE ( 'NONE', #11391, 0.1000000000000000056 ) ;
#124565=AXIS2_PLACEMENT_3D ( 'NONE', #118532, #78641, #20984 ) ;
#124566=AXIS2_PLACEMENT_3D ( 'NONE', #117760, #56278, #78531 ) ;
#124568=DIRECTION ( 'NONE',  ( 0.000000000000000000, 1.000000000000000000, 0.000000000000000000 ) ) ;
#124569=CARTESIAN_POINT ( 'NONE',  ( 1.699999999999951994, 2.500000000000000000, -4.330127018922201643 ) ) ;
#124570=FACE_OUTER_BOUND ( 'NONE', #118913, .T. ) ;
#124571=DIRECTION ( 'NONE',  ( 0.000000000000000000, 0.000000000000000000, 1.000000000000000000 ) ) ;
#124573=DIRECTION ( 'NONE',  ( -0.000000000000000000, 1.000000000000000000, -0.000000000000000000 ) ) ;
#124574=DIRECTION ( 'NONE',  ( 0.000000000000000000, 1.000000000000000000, 0.000000000000000000 ) ) ;
#124575=EDGE_LOOP ( 'NONE', ( #64324, #93353 ) ) ;
#124576=AXIS2_PLACEMENT_3D ( 'NONE', #99528, #9842, #90314 ) ;
#124577=CARTESIAN_POINT ( 'NONE',  ( -7.500000000000013323, 2.500000000000000000, 5.022947341949748790 ) ) ;
#124578=EDGE_CURVE ( 'NONE', #57241, #15129, #44090, .T. ) ;
#124579=ORIENTED_EDGE ( 'NONE', *, *, #100698, .F. ) ;
#124581=DIRECTION ( 'NONE',  ( 0.000000000000000000, -0.9999939076577903929, 0.003490651415223739937 ) ) ;
#124582=CONICAL_SURFACE ( 'NONE', #68133, 0.1000000000000002554, 0.003490658503988666988 ) ;
#124583=EDGE_LOOP ( 'NONE', ( #8558, #102492, #78522, #24406 ) ) ;
#124584=DIRECTION ( 'NONE',  ( 0.000000000000000000, -0.000000000000000000, 1.000000000000000000 ) ) ;
#124585=LINE ( 'NONE', #23811, #38357 ) ;
#124586=CARTESIAN_POINT ( 'NONE',  ( 5.799999999999931433, 2.500000000000000000, 4.230127018922196669 ) ) ;
#124587=AXIS2_PLACEMENT_3D ( 'NONE', #46057, #95790, #116068 ) ;
#124588=AXIS2_PLACEMENT_3D ( 'NONE', #6105, #45415, #46059 ) ;
#124589=ORIENTED_EDGE ( 'NONE', *, *, #58409, .T. ) ;
#124590=CARTESIAN_POINT ( 'NONE',  ( 4.399999999999937295, 12.50000000000000000, 3.983716857408420964 ) ) ;
#124591=VECTOR ( 'NONE', #22236, 1000.000000000000000 ) ;
#124592=FACE_OUTER_BOUND ( 'NONE', #23523, .T. ) ;
#124593=EDGE_CURVE ( 'NONE', #120092, #82094, #77532, .T. ) ;
#124594=EDGE_CURVE ( 'NONE', #113477, #101366, #69209, .T. ) ;
#124595=ORIENTED_EDGE ( 'NONE', *, *, #61524, .F. ) ;
#124596=DIRECTION ( 'NONE',  ( -4.274815082592931898E-19, -0.9999939076577903929, -0.003490651415223739937 ) ) ;
#124597=VECTOR ( 'NONE', #79672, 1000.000000000000000 ) ;
#124598=VERTEX_POINT ( 'NONE', #122675 ) ;
#124599=VECTOR ( 'NONE', #73943, 1000.000000000000000 ) ;
#124600=CONICAL_SURFACE ( 'NONE', #68154, 0.09999999999999982514, 0.003490658503988666988 ) ;
#124601=ORIENTED_EDGE ( 'NONE', *, *, #41057, .F. ) ;
#124602=DIRECTION ( 'NONE',  ( 0.000000000000000000, 1.000000000000000000, 0.000000000000000000 ) ) ;
#124603=CARTESIAN_POINT ( 'NONE',  ( 10.64999999999990976, 2.500000000000000000, 1.818653347947321475 ) ) ;
#124604=ADVANCED_FACE ( 'NONE', ( #1603 ), #54536, .T. ) ;
#124605=ORIENTED_EDGE ( 'NONE', *, *, #20621, .F. ) ;
#124606=DIRECTION ( 'NONE',  ( 0.000000000000000000, -0.000000000000000000, 1.000000000000000000 ) ) ;
#124607=CARTESIAN_POINT ( 'NONE',  ( -13.94999999999998685, 2.500000000000000000, 1.918653347947325338 ) ) ;
#124608=VERTEX_POINT ( 'NONE', #83411 ) ;
#124609=CARTESIAN_POINT ( 'NONE',  ( -6.650000000000018119, 2.500000000000000000, -6.495190528383302464 ) ) ;
#124610=DIRECTION ( 'NONE',  ( 0.000000000000000000, 0.000000000000000000, -1.000000000000000000 ) ) ;
#124611=DIRECTION ( 'NONE',  ( 0.000000000000000000, 0.000000000000000000, 1.000000000000000000 ) ) ;
#124612=CARTESIAN_POINT ( 'NONE',  ( -11.05000000000000249, 2.500000000000000000, -1.818653347947322141 ) ) ;
#124613=FACE_OUTER_BOUND ( 'NONE', #87756, .T. ) ;
#124614=FACE_OUTER_BOUND ( 'NONE', #40186, .T. ) ;
#124615=DIRECTION ( 'NONE',  ( -0.000000000000000000, 1.000000000000000000, -0.000000000000000000 ) ) ;
#124616=ORIENTED_EDGE ( 'NONE', *, *, #129357, .F. ) ;
#124617=ORIENTED_EDGE ( 'NONE', *, *, #37917, .F. ) ;
#124618=EDGE_LOOP ( 'NONE', ( #90909, #57480, #52887, #98425 ) ) ;
#124619=ORIENTED_EDGE ( 'NONE', *, *, #13107, .T. ) ;
#124620=CARTESIAN_POINT ( 'NONE',  ( -8.550000000000009592, 2.500000000000000000, 6.941600689897073018 ) ) ;
#124621=DIRECTION ( 'NONE',  ( 0.000000000000000000, 0.000000000000000000, 1.000000000000000000 ) ) ;
#124622=FACE_OUTER_BOUND ( 'NONE', #33971, .T. ) ;
#124623=ORIENTED_EDGE ( 'NONE', *, *, #95409, .T. ) ;
#124624=FACE_BOUND ( 'NONE', #127748, .T. ) ;
#124625=DIRECTION ( 'NONE',  ( 0.000000000000000000, -0.9999939076577903929, 0.003490651415223739937 ) ) ;
#124626=CARTESIAN_POINT ( 'NONE',  ( 12.89999999999990088, 12.50000000000000000, -4.330127018922201643 ) ) ;
#124627=FACE_OUTER_BOUND ( 'NONE', #88982, .T. ) ;
#124628=EDGE_CURVE ( 'NONE', #56748, #90263, #27343, .T. ) ;
#124629=AXIS2_PLACEMENT_3D ( 'NONE', #64264, #33539, #125130 ) ;
#124630=DIRECTION ( 'NONE',  ( 0.000000000000000000, -0.000000000000000000, 1.000000000000000000 ) ) ;
#124631=CONICAL_SURFACE ( 'NONE', #43091, 0.1000000000000000056, 0.003490658503988666988 ) ;
#124632=CARTESIAN_POINT ( 'NONE',  ( 10.44999999999991402, 2.500000000000000000, -2.065063509461102065 ) ) ;
#124633=DIRECTION ( 'NONE',  ( 0.000000000000000000, -0.9999939076577903929, 0.003490651415223739937 ) ) ;
#124634=DIRECTION ( 'NONE',  ( 0.000000000000000000, -0.000000000000000000, 1.000000000000000000 ) ) ;
#124635=PLANE ( 'NONE',  #45086 ) ;
#124636=EDGE_CURVE ( 'NONE', #14824, #62384, #16952, .T. ) ;
#124637=DIRECTION ( 'NONE',  ( 0.000000000000000000, 0.000000000000000000, 1.000000000000000000 ) ) ;
#124638=ADVANCED_FACE ( 'NONE', ( #91283 ), #84026, .T. ) ;
#124639=EDGE_CURVE ( 'NONE', #72184, #60686, #110910, .T. ) ;
#124640=FACE_OUTER_BOUND ( 'NONE', #120117, .T. ) ;
#124641=CONICAL_SURFACE ( 'NONE', #45223, 0.1000000000000002554, 0.003490658503988666988 ) ;
#124642=CIRCLE ( 'NONE', #15948, 0.1000000000000002554 ) ;
#124643=ORIENTED_EDGE ( 'NONE', *, *, #82395, .F. ) ;
#124644=ORIENTED_EDGE ( 'NONE', *, *, #101931, .F. ) ;
#124645=ORIENTED_EDGE ( 'NONE', *, *, #44060, .T. ) ;
#124646=VERTEX_POINT ( 'NONE', #93228 ) ;
#124647=CARTESIAN_POINT ( 'NONE',  ( 11.04999999999991189, 2.500000000000000000, 6.248780366869521430 ) ) ;
#124648=EDGE_CURVE ( 'NONE', #95927, #32380, #92198, .T. ) ;
#124649=ORIENTED_EDGE ( 'NONE', *, *, #94508, .F. ) ;
#124650=FACE_OUTER_BOUND ( 'NONE', #35093, .T. ) ;
#124651=EDGE_CURVE ( 'NONE', #92128, #52089, #58765, .T. ) ;
#124652=EDGE_CURVE ( 'NONE', #110742, #33188, #33032, .T. ) ;
#124653=EDGE_LOOP ( 'NONE', ( #55238, #19130 ) ) ;
#124654=ORIENTED_EDGE ( 'NONE', *, *, #119489, .F. ) ;
#124655=CIRCLE ( 'NONE', #101670, 0.06509327318403745899 ) ;
#124656=AXIS2_PLACEMENT_3D ( 'NONE', #10586, #81918, #40742 ) ;
#124657=AXIS2_PLACEMENT_3D ( 'NONE', #65411, #124986, #6460 ) ;
#124658=EDGE_CURVE ( 'NONE', #39091, #115638, #72934, .T. ) ;
#124659=CARTESIAN_POINT ( 'NONE',  ( 10.64999999999991331, 2.500000000000000000, -1.918653347947325782 ) ) ;
#124660=CARTESIAN_POINT ( 'NONE',  ( -8.150000000000012790, 2.500000000000000000, 1.818653347947321475 ) ) ;
#124661=FACE_OUTER_BOUND ( 'NONE', #51648, .T. ) ;
#124662=DIRECTION ( 'NONE',  ( 0.000000000000000000, 0.000000000000000000, 1.000000000000000000 ) ) ;
#124663=EDGE_CURVE ( 'NONE', #121393, #123488, #14814, .T. ) ;
#124665=ADVANCED_FACE ( 'NONE', ( #112220 ), #121446, .T. ) ;
#124666=VERTEX_POINT ( 'NONE', #103029 ) ;
#124668=DIRECTION ( 'NONE',  ( -0.000000000000000000, 1.000000000000000000, -0.000000000000000000 ) ) ;
#124669=ORIENTED_EDGE ( 'NONE', *, *, #118706, .T. ) ;
#124670=CARTESIAN_POINT ( 'NONE',  ( 21.34481565588170326, -0.7053969147713214927, -2.184679923000713231 ) ) ;
#124672=CIRCLE ( 'NONE', #68216, 0.09999999999999982514 ) ;
#124673=ORIENTED_EDGE ( 'NONE', *, *, #48864, .F. ) ;
#124674=CARTESIAN_POINT ( 'NONE',  ( -6.850000000000013856, 2.500000000000000000, 1.818653347947321475 ) ) ;
#124675=FACE_OUTER_BOUND ( 'NONE', #69923, .T. ) ;
#124676=DIRECTION ( 'NONE',  ( 0.000000000000000000, 0.000000000000000000, 1.000000000000000000 ) ) ;
#124677=AXIS2_PLACEMENT_3D ( 'NONE', #48121, #127957, #99156 ) ;
#124678=AXIS2_PLACEMENT_3D ( 'NONE', #18593, #107620, #87318 ) ;
#124679=DIRECTION ( 'NONE',  ( 0.000000000000000000, 0.000000000000000000, -1.000000000000000000 ) ) ;
#124680=CARTESIAN_POINT ( 'NONE',  ( -7.950000000000009059, 2.500000000000000000, 6.395190528383296602 ) ) ;
#124681=AXIS2_PLACEMENT_3D ( 'NONE', #106598, #26759, #37860 ) ;
#124682=CIRCLE ( 'NONE', #97566, 0.06509327318403745899 ) ;
#124683=ORIENTED_EDGE ( 'NONE', *, *, #86694, .T. ) ;
#124684=DIRECTION ( 'NONE',  ( -0.000000000000000000, 1.000000000000000000, -0.000000000000000000 ) ) ;
#124685=ORIENTED_EDGE ( 'NONE', *, *, #17978, .T. ) ;
#124686=AXIS2_PLACEMENT_3D ( 'NONE', #116664, #17813, #18468 ) ;
#124687=CARTESIAN_POINT ( 'NONE',  ( 6.849999999999930367, 12.50000000000000000, -6.213873640053564351 ) ) ;
#124688=ORIENTED_EDGE ( 'NONE', *, *, #92897, .F. ) ;
#124689=CARTESIAN_POINT ( 'NONE',  ( 11.64999999999990266, 2.500000000000000000, 2.165063509461097713 ) ) ;
#124690=CARTESIAN_POINT ( 'NONE',  ( 10.39999999999990976, 2.500000000000000000, -4.330127018922201643 ) ) ;
#124691=CARTESIAN_POINT ( 'NONE',  ( -7.499999999999980460, 2.500000000000000000, -2.276824562219559311E-15 ) ) ;
#124692=DIRECTION ( 'NONE',  ( 0.000000000000000000, 0.000000000000000000, -1.000000000000000000 ) ) ;
#124693=ORIENTED_EDGE ( 'NONE', *, *, #15711, .F. ) ;
#124694=AXIS2_PLACEMENT_3D ( 'NONE', #41065, #104929, #104307 ) ;
#124695=ADVANCED_FACE ( 'NONE', ( #52639 ), #92575, .T. ) ;
#124696=AXIS2_PLACEMENT_3D ( 'NONE', #31309, #13565, #71204 ) ;
#124697=DIRECTION ( 'NONE',  ( 0.000000000000000000, 0.000000000000000000, 1.000000000000000000 ) ) ;
#124698=EDGE_CURVE ( 'NONE', #9617, #106262, #62959, .T. ) ;
#124699=VERTEX_POINT ( 'NONE', #106887 ) ;
#124700=VERTEX_POINT ( 'NONE', #6106 ) ;
#124701=EDGE_LOOP ( 'NONE', ( #114299, #107814 ) ) ;
#124702=DIRECTION ( 'NONE',  ( -0.000000000000000000, -1.000000000000000000, -0.000000000000000000 ) ) ;
#124703=DIRECTION ( 'NONE',  ( -0.000000000000000000, 1.000000000000000000, -0.000000000000000000 ) ) ;
#124705=DIRECTION ( 'NONE',  ( -0.000000000000000000, -1.000000000000000000, -0.000000000000000000 ) ) ;
#124706=DIRECTION ( 'NONE',  ( -0.000000000000000000, -1.000000000000000000, -0.000000000000000000 ) ) ;
#124707=LINE ( 'NONE', #46139, #98855 ) ;
#124708=ORIENTED_EDGE ( 'NONE', *, *, #95400, .T. ) ;
#124709=CARTESIAN_POINT ( 'NONE',  ( -12.29999999999999538, 2.500000000000000000, -4.676537180435976104 ) ) ;
#124710=ORIENTED_EDGE ( 'NONE', *, *, #39050, .F. ) ;
#124711=DIRECTION ( 'NONE',  ( 0.000000000000000000, 0.000000000000000000, -1.000000000000000000 ) ) ;
#124712=LINE ( 'NONE', #64498, #75613 ) ;
#124713=LINE ( 'NONE', #104425, #46006 ) ;
#124714=EDGE_LOOP ( 'NONE', ( #129425, #4854, #15021, #2332 ) ) ;
#124715=CIRCLE ( 'NONE', #68271, 0.1000000000000000056 ) ;
#124716=CIRCLE ( 'NONE', #105844, 0.1000000000000002554 ) ;
#124717=DIRECTION ( 'NONE',  ( -0.000000000000000000, -1.000000000000000000, -0.000000000000000000 ) ) ;
#124718=DIRECTION ( 'NONE',  ( 0.000000000000000000, 0.000000000000000000, -1.000000000000000000 ) ) ;
#124719=ORIENTED_EDGE ( 'NONE', *, *, #57897, .F. ) ;
#124720=CIRCLE ( 'NONE', #47368, 0.06509327318403745899 ) ;
#124721=AXIS2_PLACEMENT_3D ( 'NONE', #36404, #8668, #39477 ) ;
#124722=DIRECTION ( 'NONE',  ( 0.000000000000000000, 0.000000000000000000, 1.000000000000000000 ) ) ;
#124723=EDGE_CURVE ( 'NONE', #21305, #46048, #56502, .T. ) ;
#124724=ORIENTED_EDGE ( 'NONE', *, *, #127470, .F. ) ;
#124725=EDGE_LOOP ( 'NONE', ( #32273, #128729 ) ) ;
#124726=DIRECTION ( 'NONE',  ( 0.000000000000000000, 0.000000000000000000, -1.000000000000000000 ) ) ;
#124727=EDGE_LOOP ( 'NONE', ( #28959, #38448, #110541, #7657, #27741, #123100, #36931, #115364, #104668, #7427, #117444, #80057, #128536 ) ) ;
#124728=CARTESIAN_POINT ( 'NONE',  ( 18.27284318114930883, 0.4998542452743989783, -4.791717918552158118 ) ) ;
#124729=DIRECTION ( 'NONE',  ( -0.000000000000000000, 1.000000000000000000, -0.000000000000000000 ) ) ;
#124730=CIRCLE ( 'NONE', #66236, 0.06509327318403745899 ) ;
#124732=CARTESIAN_POINT ( 'NONE',  ( -11.84999999999999609, 2.500000000000000000, 6.941600689897073018 ) ) ;
#124733=EDGE_CURVE ( 'NONE', #56716, #69025, #98452, .T. ) ;
#124734=ORIENTED_EDGE ( 'NONE', *, *, #36983, .F. ) ;
#124735=CIRCLE ( 'NONE', #53634, 0.1000000000000002554 ) ;
#124736=FACE_BOUND ( 'NONE', #10558, .T. ) ;
#124737=CARTESIAN_POINT ( 'NONE',  ( -6.071532165918824830E-15, 12.50000000000000000, -4.330127018922201643 ) ) ;
#124738=DIRECTION ( 'NONE',  ( 0.000000000000000000, 0.000000000000000000, -1.000000000000000000 ) ) ;
#124739=ORIENTED_EDGE ( 'NONE', *, *, #119584, .T. ) ;
#124740=EDGE_CURVE ( 'NONE', #30745, #70927, #113133, .T. ) ;
#124741=CARTESIAN_POINT ( 'NONE',  ( -11.24999999999996447, 12.50000000000000000, -6.495190528383298911 ) ) ;
#124742=DIRECTION ( 'NONE',  ( -0.000000000000000000, 1.000000000000000000, -0.000000000000000000 ) ) ;
#124743=ADVANCED_FACE ( 'NONE', ( #66955 ), #90129, .T. ) ;
#124744=ORIENTED_EDGE ( 'NONE', *, *, #94762, .F. ) ;
#124745=ORIENTED_EDGE ( 'NONE', *, *, #55792, .T. ) ;
#124746=ADVANCED_FACE ( 'NONE', ( #76160 ), #106859, .T. ) ;
#124747=ORIENTED_EDGE ( 'NONE', *, *, #44060, .F. ) ;
#124748=CARTESIAN_POINT ( 'NONE',  ( -3.550000000000028244, 2.500000000000000000, 2.611473670974873151 ) ) ;
#124749=DIRECTION ( 'NONE',  ( -0.000000000000000000, 1.000000000000000000, -0.000000000000000000 ) ) ;
#124750=CARTESIAN_POINT ( 'NONE',  ( 7.099999999999928590, 2.500000000000000000, 3.637306695894644726 ) ) ;
#124751=EDGE_CURVE ( 'NONE', #62839, #101653, #33720, .T. ) ;
#124752=FACE_BOUND ( 'NONE', #2748, .T. ) ;
#124753=VERTEX_POINT ( 'NONE', #35596 ) ;
#124754=AXIS2_PLACEMENT_3D ( 'NONE', #109680, #20014, #49486 ) ;
#124756=CONICAL_SURFACE ( 'NONE', #68316, 0.09999999999999982514, 0.003490658503988666988 ) ;
#124757=CARTESIAN_POINT ( 'NONE',  ( -0.4500000000000397571, 2.500000000000000000, -6.595190528383302109 ) ) ;
#124758=CARTESIAN_POINT ( 'NONE',  ( -11.64999999999999680, 2.500000000000000000, 2.165063509461097713 ) ) ;
#124759=CARTESIAN_POINT ( 'NONE',  ( -11.05000000000000071, 2.500000000000000000, 2.511473670974873507 ) ) ;
#124760=AXIS2_PLACEMENT_3D ( 'NONE', #68234, #67581, #97059 ) ;
#124761=CARTESIAN_POINT ( 'NONE',  ( -1.450000000000035927, 2.500000000000000000, -1.818653347947326138 ) ) ;
#124762=PLANE ( 'NONE',  #8905 ) ;
#124763=DIRECTION ( 'NONE',  ( -0.000000000000000000, 1.000000000000000000, -0.000000000000000000 ) ) ;
#124764=VECTOR ( 'NONE', #62654, 1000.000000000000000 ) ;
#124765=CARTESIAN_POINT ( 'NONE',  ( 7.699999999999923794, 2.500000000000000000, -3.983716857408426293 ) ) ;
#124766=CIRCLE ( 'NONE', #7673, 0.1000000000000002554 ) ;
#124767=CARTESIAN_POINT ( 'NONE',  ( -10.00000000000000355, 2.500000000000000000, -0.5928203230275541635 ) ) ;
#124768=AXIS2_PLACEMENT_3D ( 'NONE', #113943, #34098, #72731 ) ;
#124769=EDGE_LOOP ( 'NONE', ( #70907, #57895 ) ) ;
#124770=ORIENTED_EDGE ( 'NONE', *, *, #75697, .F. ) ;
#124771=EDGE_LOOP ( 'NONE', ( #55348, #20749 ) ) ;
#124772=ORIENTED_EDGE ( 'NONE', *, *, #123572, .T. ) ;
#124773=ORIENTED_EDGE ( 'NONE', *, *, #114163, .F. ) ;
#124774=DIRECTION ( 'NONE',  ( 0.000000000000000000, 0.000000000000000000, -1.000000000000000000 ) ) ;
#124775=DIRECTION ( 'NONE',  ( -4.274815082592931898E-19, -0.9999939076577903929, -0.003490651415223739937 ) ) ;
#124776=AXIS2_PLACEMENT_3D ( 'NONE', #112589, #21623, #92279 ) ;
#124777=ORIENTED_EDGE ( 'NONE', *, *, #61415, .F. ) ;
#124778=FACE_BOUND ( 'NONE', #36523, .T. ) ;
#124779=VECTOR ( 'NONE', #89177, 1000.000000000000000 ) ;
#124780=CARTESIAN_POINT ( 'NONE',  ( 1.049999999999954525, 12.50000000000000000, 1.883746621131358934 ) ) ;
#124781=ADVANCED_FACE ( 'NONE', ( #86608 ), #86019, .T. ) ;
#124782=AXIS2_PLACEMENT_3D ( 'NONE', #95368, #67153, #106465 ) ;
#124783=CIRCLE ( 'NONE', #22391, 0.1000000000000000472 ) ;
#124785=ORIENTED_EDGE ( 'NONE', *, *, #124651, .F. ) ;
#124786=LINE ( 'NONE', #42364, #47412 ) ;
#124788=EDGE_CURVE ( 'NONE', #27686, #118657, #344, .T. ) ;
#124789=DIRECTION ( 'NONE',  ( 0.000000000000000000, -0.000000000000000000, 1.000000000000000000 ) ) ;
#124790=ORIENTED_EDGE ( 'NONE', *, *, #124002, .T. ) ;
#124792=EDGE_CURVE ( 'NONE', #6072, #50160, #117302, .T. ) ;
#124793=ORIENTED_EDGE ( 'NONE', *, *, #86183, .T. ) ;
#124794=ORIENTED_EDGE ( 'NONE', *, *, #118587, .F. ) ;
#124795=EDGE_LOOP ( 'NONE', ( #49335, #52145, #115191, #17086 ) ) ;
#124796=EDGE_CURVE ( 'NONE', #115621, #41467, #94343, .T. ) ;
#124797=PLANE ( 'NONE',  #2786 ) ;
#124798=DIRECTION ( 'NONE',  ( -4.274815082592931898E-19, -0.9999939076577903929, -0.003490651415223739937 ) ) ;
#124799=EDGE_CURVE ( 'NONE', #125318, #46605, #81827, .T. ) ;
#124800=FACE_OUTER_BOUND ( 'NONE', #45142, .T. ) ;
#124801=ADVANCED_FACE ( 'NONE', ( #66325 ), #54635, .T. ) ;
#124802=ORIENTED_EDGE ( 'NONE', *, *, #77336, .T. ) ;
#124803=CIRCLE ( 'NONE', #76684, 0.06509327318403745899 ) ;
#124804=CARTESIAN_POINT ( 'NONE',  ( 4.912722231824622199, 1.499999999999620082, -9.942384337864433874 ) ) ;
#124805=EDGE_CURVE ( 'NONE', #126729, #69733, #54563, .T. ) ;
#124806=CARTESIAN_POINT ( 'NONE',  ( -8.150000000000009237, 2.500000000000000000, 6.248780366869520542 ) ) ;
#124807=CARTESIAN_POINT ( 'NONE',  ( -7.300000000000013145, 2.500000000000000000, 4.083716857408420609 ) ) ;
#124811=DIRECTION ( 'NONE',  ( 0.000000000000000000, -0.000000000000000000, 1.000000000000000000 ) ) ;
#124812=ORIENTED_EDGE ( 'NONE', *, *, #16190, .T. ) ;
#124813=DIRECTION ( 'NONE',  ( 0.000000000000000000, 0.000000000000000000, -1.000000000000000000 ) ) ;
#124814=EDGE_CURVE ( 'NONE', #49458, #96815, #29602, .T. ) ;
#124815=EDGE_CURVE ( 'NONE', #10654, #57940, #19116, .T. ) ;
#124817=ORIENTED_EDGE ( 'NONE', *, *, #125113, .F. ) ;
#124818=AXIS2_PLACEMENT_3D ( 'NONE', #30071, #89619, #69987 ) ;
#124819=VERTEX_POINT ( 'NONE', #95154 ) ;
#124822=FACE_OUTER_BOUND ( 'NONE', #116877, .T. ) ;
#124823=CARTESIAN_POINT ( 'NONE',  ( 10.64999999999990976, 2.500000000000000000, 1.918653347947321564 ) ) ;
#124825=ORIENTED_EDGE ( 'NONE', *, *, #33906, .F. ) ;
#124826=AXIS2_PLACEMENT_3D ( 'NONE', #11039, #19589, #69983 ) ;
#124827=ORIENTED_EDGE ( 'NONE', *, *, #55054, .F. ) ;
#124828=LINE ( 'NONE', #3755, #20411 ) ;
#124829=DIRECTION ( 'NONE',  ( 0.000000000000000000, 0.000000000000000000, -1.000000000000000000 ) ) ;
#124830=CARTESIAN_POINT ( 'NONE',  ( -11.24999999999996447, 2.500000000000000000, -2.165063509461097713 ) ) ;
#124831=ORIENTED_EDGE ( 'NONE', *, *, #78851, .F. ) ;
#124832=ORIENTED_EDGE ( 'NONE', *, *, #12389, .F. ) ;
#124833=CARTESIAN_POINT ( 'NONE',  ( 8.949999999999917577, 2.500000000000000000, -2.511473670974877948 ) ) ;
#124834=AXIS2_PLACEMENT_3D ( 'NONE', #29889, #54993, #58706 ) ;
#124835=ORIENTED_EDGE ( 'NONE', *, *, #42959, .T. ) ;
#124836=CARTESIAN_POINT ( 'NONE',  ( -8.950000000000009948, 12.50000000000000000, -6.906693963081109722 ) ) ;
#124837=VECTOR ( 'NONE', #53314, 1000.000000000000000 ) ;
#124838=DIRECTION ( 'NONE',  ( -0.000000000000000000, -1.000000000000000000, -0.000000000000000000 ) ) ;
#124839=VERTEX_POINT ( 'NONE', #76804 ) ;
#124840=DIRECTION ( 'NONE',  ( -4.274815082592931898E-19, -0.9999939076577903929, -0.003490651415223739937 ) ) ;
#124841=FACE_OUTER_BOUND ( 'NONE', #89338, .T. ) ;
#124842=DIRECTION ( 'NONE',  ( 0.000000000000000000, 1.000000000000000000, 0.000000000000000000 ) ) ;
#124843=DIRECTION ( 'NONE',  ( -0.000000000000000000, 1.000000000000000000, -0.000000000000000000 ) ) ;
#124844=ORIENTED_EDGE ( 'NONE', *, *, #89676, .F. ) ;
#124845=CARTESIAN_POINT ( 'NONE',  ( 1.649999999999951061, 2.500000000000000000, -6.495190528383302464 ) ) ;
#124846=EDGE_CURVE ( 'NONE', #41921, #64447, #113220, .T. ) ;
#124848=ORIENTED_EDGE ( 'NONE', *, *, #117971, .T. ) ;
#124849=ORIENTED_EDGE ( 'NONE', *, *, #50894, .T. ) ;
#124850=DIRECTION ( 'NONE',  ( 0.000000000000000000, -0.9999939076577903929, 0.003490651415223739937 ) ) ;
#124851=FACE_OUTER_BOUND ( 'NONE', #50745, .T. ) ;
#124852=DIRECTION ( 'NONE',  ( 0.000000000000000000, 0.000000000000000000, 1.000000000000000000 ) ) ;
#124853=AXIS2_PLACEMENT_3D ( 'NONE', #18380, #19013, #127692 ) ;
#124854=DIRECTION ( 'NONE',  ( -0.000000000000000000, 1.000000000000000000, -0.000000000000000000 ) ) ;
#124855=CIRCLE ( 'NONE', #99729, 0.1000000000000000472 ) ;
#124856=DIRECTION ( 'NONE',  ( 0.000000000000000000, 0.000000000000000000, 1.000000000000000000 ) ) ;
#124857=EDGE_CURVE ( 'NONE', #4381, #79978, #46323, .T. ) ;
#124858=DIRECTION ( 'NONE',  ( 0.000000000000000000, 0.000000000000000000, -1.000000000000000000 ) ) ;
#124859=FACE_OUTER_BOUND ( 'NONE', #46642, .T. ) ;
#124860=CARTESIAN_POINT ( 'NONE',  ( -10.20000000000000284, 12.50000000000000000, 3.983716857408420964 ) ) ;
#124861=CARTESIAN_POINT ( 'NONE',  ( -12.69999999999999396, 12.50000000000000000, -3.918623584224386391 ) ) ;
#124862=CIRCLE ( 'NONE', #20402, 0.09999999999999982514 ) ;
#124863=VECTOR ( 'NONE', #53478, 1000.000000000000000 ) ;
#124864=DIRECTION ( 'NONE',  ( -0.000000000000000000, 1.000000000000000000, -0.000000000000000000 ) ) ;
#124865=ORIENTED_EDGE ( 'NONE', *, *, #69303, .T. ) ;
#124866=VERTEX_POINT ( 'NONE', #8045 ) ;
#124867=CIRCLE ( 'NONE', #122806, 0.1000000000000000472 ) ;
#124868=CIRCLE ( 'NONE', #101880, 0.09999999999999982514 ) ;
#124869=VERTEX_POINT ( 'NONE', #28999 ) ;
#124870=ORIENTED_EDGE ( 'NONE', *, *, #53385, .F. ) ;
#124871=CIRCLE ( 'NONE', #39222, 0.09999999999999982514 ) ;
#124872=LINE ( 'NONE', #14875, #39459 ) ;
#124873=DIRECTION ( 'NONE',  ( 0.000000000000000000, 0.000000000000000000, -1.000000000000000000 ) ) ;
#124874=DIRECTION ( 'NONE',  ( 0.000000000000000000, 1.000000000000000000, 0.000000000000000000 ) ) ;
#124875=VERTEX_POINT ( 'NONE', #119291 ) ;
#124876=CARTESIAN_POINT ( 'NONE',  ( -0.2000000000000404232, 2.500000000000000000, 3.983716857408420964 ) ) ;
#124877=CIRCLE ( 'NONE', #122816, 0.06509327318403745899 ) ;
#124878=AXIS2_PLACEMENT_3D ( 'NONE', #71840, #113695, #44295 ) ;
#124879=DIRECTION ( 'NONE',  ( 0.000000000000000000, -0.9999939076577903929, 0.003490651415223739937 ) ) ;
#124880=CARTESIAN_POINT ( 'NONE',  ( -10.00000000000000711, 2.500000000000000000, -3.637306695894645614 ) ) ;
#124881=EDGE_LOOP ( 'NONE', ( #90664, #102078 ) ) ;
#124882=DIRECTION ( 'NONE',  ( 0.000000000000000000, 1.000000000000000000, 0.000000000000000000 ) ) ;
#124883=ORIENTED_EDGE ( 'NONE', *, *, #124892, .F. ) ;
#124884=VERTEX_POINT ( 'NONE', #17868 ) ;
#124885=ORIENTED_EDGE ( 'NONE', *, *, #22829, .F. ) ;
#124886=VERTEX_POINT ( 'NONE', #119950 ) ;
#124887=LINE ( 'NONE', #125519, #103265 ) ;
#124888=AXIS2_PLACEMENT_3D ( 'NONE', #36213, #128468, #96392 ) ;
#124889=CARTESIAN_POINT ( 'NONE',  ( -14.99999999999998401, 2.500000000000000000, 0.6928203230275518099 ) ) ;
#124890=PLANE ( 'NONE',  #56666 ) ;
#124891=CARTESIAN_POINT ( 'NONE',  ( 5.849999999999933920, 2.500000000000000000, -2.857883832488653741 ) ) ;
#124892=EDGE_CURVE ( 'NONE', #2147, #84545, #4437, .T. ) ;
#124893=VERTEX_POINT ( 'NONE', #128506 ) ;
#124894=DIRECTION ( 'NONE',  ( 0.000000000000000000, 0.000000000000000000, 1.000000000000000000 ) ) ;
#124895=ORIENTED_EDGE ( 'NONE', *, *, #20445, .F. ) ;
#124896=CARTESIAN_POINT ( 'NONE',  ( 81.97620568616159176, -3.937821671072774699, -6.124242985517362570 ) ) ;
#124897=CARTESIAN_POINT ( 'NONE',  ( 3.710216157319379260, -2.499999999999999556, -9.999999999879436885 ) ) ;
#124898=EDGE_CURVE ( 'NONE', #77184, #61867, #49940, .T. ) ;
#124899=EDGE_CURVE ( 'NONE', #67339, #60096, #121531, .T. ) ;
#124900=CARTESIAN_POINT ( 'NONE',  ( -8.350000000000013856, 2.500000000000000000, -5.902370205355745192 ) ) ;
#124901=FACE_OUTER_BOUND ( 'NONE', #70607, .T. ) ;
#124902=EDGE_CURVE ( 'NONE', #97917, #76656, #108819, .T. ) ;
#124903=ORIENTED_EDGE ( 'NONE', *, *, #20870, .T. ) ;
#124904=AXIS2_PLACEMENT_3D ( 'NONE', #121929, #93123, #91177 ) ;
#124905=ORIENTED_EDGE ( 'NONE', *, *, #128652, .T. ) ;
#124906=ADVANCED_FACE ( 'NONE', ( #38841 ), #23328, .T. ) ;
#124907=ORIENTED_EDGE ( 'NONE', *, *, #54934, .T. ) ;
#124908=DIRECTION ( 'NONE',  ( 0.000000000000000000, 1.000000000000000000, 0.000000000000000000 ) ) ;
#124909=CARTESIAN_POINT ( 'NONE',  ( -8.150000000000009237, 12.50000000000000000, 6.906693963081109722 ) ) ;
#124910=FACE_OUTER_BOUND ( 'NONE', #16305, .T. ) ;
#124911=EDGE_CURVE ( 'NONE', #84876, #86058, #17038, .T. ) ;
#124912=FACE_BOUND ( 'NONE', #9354, .T. ) ;
#124913=CARTESIAN_POINT ( 'NONE',  ( 5.199999999999937117, 2.500000000000000000, -4.676537180435978769 ) ) ;
#124914=DIRECTION ( 'NONE',  ( 0.000000000000000000, 0.000000000000000000, 1.000000000000000000 ) ) ;
#124915=VECTOR ( 'NONE', #6372, 1000.000000000000000 ) ;
#124916=AXIS2_PLACEMENT_3D ( 'NONE', #126163, #75761, #124237 ) ;
#124917=FACE_OUTER_BOUND ( 'NONE', #89275, .T. ) ;
#124918=CONICAL_SURFACE ( 'NONE', #20367, 0.1000000000000000472, 0.003490658503988666988 ) ;
#124920=DIRECTION ( 'NONE',  ( -0.000000000000000000, -1.000000000000000000, -0.000000000000000000 ) ) ;
#124921=DIRECTION ( 'NONE',  ( 0.000000000000000000, 0.000000000000000000, 1.000000000000000000 ) ) ;
#124922=ORIENTED_EDGE ( 'NONE', *, *, #129542, .F. ) ;
#124923=CIRCLE ( 'NONE', #5684, 0.1000000000000002554 ) ;
#124924=FACE_OUTER_BOUND ( 'NONE', #106939, .T. ) ;
#124925=ORIENTED_EDGE ( 'NONE', *, *, #46150, .T. ) ;
#124926=EDGE_LOOP ( 'NONE', ( #59770, #8389, #119491, #11917 ) ) ;
#124927=EDGE_LOOP ( 'NONE', ( #74068, #87749, #103069, #93415 ) ) ;
#124928=ORIENTED_EDGE ( 'NONE', *, *, #71669, .F. ) ;
#124929=LINE ( 'NONE', #15602, #63233 ) ;
#124930=FACE_BOUND ( 'NONE', #27863, .T. ) ;
#124931=DIRECTION ( 'NONE',  ( 0.000000000000000000, 1.000000000000000000, 0.000000000000000000 ) ) ;
#124932=CIRCLE ( 'NONE', #16147, 0.06509327318403745899 ) ;
#124933=VECTOR ( 'NONE', #26459, 1000.000000000000000 ) ;
#124934=ORIENTED_EDGE ( 'NONE', *, *, #50456, .T. ) ;
#124935=CARTESIAN_POINT ( 'NONE',  ( 34.93074629416359755, 2.900242961790199026, 4.640733549230978916 ) ) ;
#124936=CARTESIAN_POINT ( 'NONE',  ( 0.1999999999999636513, 2.500000000000000000, -0.3464101615137760715 ) ) ;
#124937=AXIS2_PLACEMENT_3D ( 'NONE', #120305, #110476, #31295 ) ;
#124938=ORIENTED_EDGE ( 'NONE', *, *, #8869, .F. ) ;
#124940=VECTOR ( 'NONE', #436, 1000.000000000000000 ) ;
#124941=CARTESIAN_POINT ( 'NONE',  ( 3.099999999999945022, 2.500000000000000000, -0.2464101615137783419 ) ) ;
#124942=AXIS2_PLACEMENT_3D ( 'NONE', #48752, #47454, #88660 ) ;
#124943=EDGE_CURVE ( 'NONE', #72947, #37042, #127804, .T. ) ;
#124944=EDGE_LOOP ( 'NONE', ( #57634, #50119, #88946, #93300 ) ) ;
#124945=ADVANCED_FACE ( 'NONE', ( #80018 ), #21195, .T. ) ;
#124946=DIRECTION ( 'NONE',  ( -0.000000000000000000, 1.000000000000000000, -0.000000000000000000 ) ) ;
#124947=DIRECTION ( 'NONE',  ( -4.274815082592931898E-19, -0.9999939076577903929, -0.003490651415223739937 ) ) ;
#124948=CONICAL_SURFACE ( 'NONE', #116624, 0.09999999999999982514, 0.003490658503988666988 ) ;
#124949=ADVANCED_FACE ( 'NONE', ( #117327 ), #27441, .T. ) ;
#124950=VECTOR ( 'NONE', #10173, 1000.000000000000000 ) ;
#124951=ORIENTED_EDGE ( 'NONE', *, *, #71618, .F. ) ;
#124952=CONICAL_SURFACE ( 'NONE', #129193, 0.1000000000000002554, 0.003490658503988666988 ) ;
#124953=CARTESIAN_POINT ( 'NONE',  ( 9.149999999999915090, 12.50000000000000000, -2.165063509461101710 ) ) ;
#124955=CARTESIAN_POINT ( 'NONE',  ( -1.450000000000035483, 2.500000000000000000, 1.818653347947321475 ) ) ;
#124956=EDGE_CURVE ( 'NONE', #48671, #74924, #58855, .T. ) ;
#124957=EDGE_LOOP ( 'NONE', ( #36890, #29723, #50720, #24404 ) ) ;
#124958=ORIENTED_EDGE ( 'NONE', *, *, #51074, .T. ) ;
#124959=AXIS2_PLACEMENT_3D ( 'NONE', #77007, #116916, #27252 ) ;
#124960=CARTESIAN_POINT ( 'NONE',  ( -0.4000000000000404898, 2.500000000000000000, 4.922947341949748257 ) ) ;
#124961=EDGE_LOOP ( 'NONE', ( #90087, #29666, #67665, #27731 ) ) ;
#124962=FACE_OUTER_BOUND ( 'NONE', #21715, .T. ) ;
#124963=LINE ( 'NONE', #105324, #87118 ) ;
#124964=EDGE_CURVE ( 'NONE', #11186, #53658, #119480, .T. ) ;
#124965=AXIS2_PLACEMENT_3D ( 'NONE', #110817, #101004, #13254 ) ;
#124966=CIRCLE ( 'NONE', #93573, 0.1000000000000002554 ) ;
#124967=EDGE_CURVE ( 'NONE', #67282, #88347, #83878, .T. ) ;
#124968=ORIENTED_EDGE ( 'NONE', *, *, #13458, .T. ) ;
#124970=CARTESIAN_POINT ( 'NONE',  ( -5.600000000000023626, 2.500000000000000000, -3.883716857408426648 ) ) ;
#124971=CARTESIAN_POINT ( 'NONE',  ( -11.64999999999999680, 2.500000000000000000, 1.472243186433545459 ) ) ;
#124972=DIRECTION ( 'NONE',  ( 0.000000000000000000, 0.000000000000000000, 1.000000000000000000 ) ) ;
#124973=DIRECTION ( 'NONE',  ( -0.000000000000000000, -1.000000000000000000, -0.000000000000000000 ) ) ;
#124974=EDGE_CURVE ( 'NONE', #59702, #41439, #69298, .T. ) ;
#124975=EDGE_LOOP ( 'NONE', ( #112288, #124141, #6525, #65746 ) ) ;
#124976=ORIENTED_EDGE ( 'NONE', *, *, #61463, .T. ) ;
#124977=CARTESIAN_POINT ( 'NONE',  ( -9.200000000000006395, 2.500000000000000000, 4.330127018922196314 ) ) ;
#124978=DIRECTION ( 'NONE',  ( 0.000000000000000000, 1.000000000000000000, 0.000000000000000000 ) ) ;
#124979=DIRECTION ( 'NONE',  ( -0.000000000000000000, 1.000000000000000000, -0.000000000000000000 ) ) ;
#124980=VERTEX_POINT ( 'NONE', #48631 ) ;
#124981=ORIENTED_EDGE ( 'NONE', *, *, #120603, .F. ) ;
#124982=ORIENTED_EDGE ( 'NONE', *, *, #53322, .F. ) ;
#124983=CARTESIAN_POINT ( 'NONE',  ( -1.450000000000035483, 2.500000000000000000, 6.148780366869520897 ) ) ;
#124984=CARTESIAN_POINT ( 'NONE',  ( -8.350000000000012079, 12.50000000000000000, -1.407149913249512663 ) ) ;
#124985=PLANE ( 'NONE',  #66439 ) ;
#124986=DIRECTION ( 'NONE',  ( -0.000000000000000000, 1.000000000000000000, -0.000000000000000000 ) ) ;
#124987=DIRECTION ( 'NONE',  ( -0.000000000000000000, -1.000000000000000000, -0.000000000000000000 ) ) ;
#124988=CARTESIAN_POINT ( 'NONE',  ( 5.849999999999933920, 2.500000000000000000, -2.065063509461102065 ) ) ;
#124989=DIRECTION ( 'NONE',  ( -0.000000000000000000, 1.000000000000000000, -0.000000000000000000 ) ) ;
#124990=DIRECTION ( 'NONE',  ( 0.000000000000000000, 0.000000000000000000, -1.000000000000000000 ) ) ;
#124991=VECTOR ( 'NONE', #65207, 1000.000000000000000 ) ;
#124992=CARTESIAN_POINT ( 'NONE',  ( -3.950000000000026379, 2.500000000000000000, -1.718653347947326049 ) ) ;
#124993=CONICAL_SURFACE ( 'NONE', #93689, 0.09999999999999982514, 0.003490658503988666988 ) ;
#124994=ORIENTED_EDGE ( 'NONE', *, *, #66425, .T. ) ;
#124995=VECTOR ( 'NONE', #29579, 1000.000000000000000 ) ;
#124996=DIRECTION ( 'NONE',  ( 0.000000000000000000, 1.000000000000000000, 0.000000000000000000 ) ) ;
#124997=ORIENTED_EDGE ( 'NONE', *, *, #20448, .T. ) ;
#124998=EDGE_LOOP ( 'NONE', ( #65320, #42041 ) ) ;
#124999=FACE_OUTER_BOUND ( 'NONE', #43606, .T. ) ;
#125000=DIRECTION ( 'NONE',  ( 0.000000000000000000, 0.000000000000000000, -1.000000000000000000 ) ) ;
#125001=FACE_OUTER_BOUND ( 'NONE', #114821, .T. ) ;
#125002=CIRCLE ( 'NONE', #70622, 0.06509327318403745899 ) ;
#125003=DIRECTION ( 'NONE',  ( 0.000000000000000000, 0.000000000000000000, -1.000000000000000000 ) ) ;
#125004=EDGE_CURVE ( 'NONE', #22231, #56350, #89195, .T. ) ;
#125005=CIRCLE ( 'NONE', #14269, 0.09999999999999982514 ) ;
#125006=CARTESIAN_POINT ( 'NONE',  ( 2.099999999999950351, 2.500000000000000000, -4.230127018922201998 ) ) ;
#125007=DIRECTION ( 'NONE',  ( 0.000000000000000000, -0.000000000000000000, 1.000000000000000000 ) ) ;
#125008=CARTESIAN_POINT ( 'NONE',  ( -5.400000000000019895, 12.50000000000000000, 3.637306695894644726 ) ) ;
#125009=EDGE_LOOP ( 'NONE', ( #93900, #61589 ) ) ;
#125010=DIRECTION ( 'NONE',  ( -0.000000000000000000, -1.000000000000000000, -0.000000000000000000 ) ) ;
#125011=LINE ( 'NONE', #94911, #70786 ) ;
#125012=ORIENTED_EDGE ( 'NONE', *, *, #107595, .F. ) ;
#125013=AXIS2_PLACEMENT_3D ( 'NONE', #70694, #10475, #31426 ) ;
#125014=ORIENTED_EDGE ( 'NONE', *, *, #9778, .F. ) ;
#125015=EDGE_LOOP ( 'NONE', ( #128916, #73688 ) ) ;
#125016=VECTOR ( 'NONE', #80110, 1000.000000000000000 ) ;
#125017=VERTEX_POINT ( 'NONE', #109484 ) ;
#125018=FACE_OUTER_BOUND ( 'NONE', #24935, .T. ) ;
#125019=PLANE ( 'NONE',  #60370 ) ;
#125020=AXIS2_PLACEMENT_3D ( 'NONE', #88852, #29942, #69196 ) ;
#125021=DIRECTION ( 'NONE',  ( -0.000000000000000000, -1.000000000000000000, -0.000000000000000000 ) ) ;
#125022=CARTESIAN_POINT ( 'NONE',  ( 5.399999999999936406, 12.50000000000000000, -5.088040615133791356 ) ) ;
#125023=AXIS2_PLACEMENT_3D ( 'NONE', #88594, #127240, #58510 ) ;
#125024=LINE ( 'NONE', #75273, #70183 ) ;
#125025=ORIENTED_EDGE ( 'NONE', *, *, #38919, .T. ) ;
#125026=DIRECTION ( 'NONE',  ( -0.000000000000000000, 1.000000000000000000, -0.000000000000000000 ) ) ;
#125027=FACE_OUTER_BOUND ( 'NONE', #77226, .T. ) ;
#125028=LINE ( 'NONE', #27454, #8085 ) ;
#125029=EDGE_LOOP ( 'NONE', ( #61271, #17108, #129173, #98486 ) ) ;
#125030=AXIS2_PLACEMENT_3D ( 'NONE', #96374, #66917, #78043 ) ;
#125031=ORIENTED_EDGE ( 'NONE', *, *, #40572, .F. ) ;
#125032=EDGE_LOOP ( 'NONE', ( #49728, #10133 ) ) ;
#125033=CARTESIAN_POINT ( 'NONE',  ( 5.849999999999933920, 12.50000000000000000, 6.430097255199259010 ) ) ;
#125034=CIRCLE ( 'NONE', #70657, 0.1000000000000002554 ) ;
#125035=DIRECTION ( 'NONE',  ( -0.000000000000000000, -1.000000000000000000, -0.000000000000000000 ) ) ;
#125036=CARTESIAN_POINT ( 'NONE',  ( -6.650000000000014566, 2.500000000000000000, 1.572243186433545548 ) ) ;
#125037=ADVANCED_FACE ( 'NONE', ( #59763 ), #100312, .T. ) ;
#125038=EDGE_LOOP ( 'NONE', ( #120620, #114321, #44803, #91857 ) ) ;
#125039=LINE ( 'NONE', #72095, #5486 ) ;
#125040=CARTESIAN_POINT ( 'NONE',  ( 0.8499999999999550138, 12.50000000000000000, -5.737276932171712751 ) ) ;
#125042=ADVANCED_FACE ( 'NONE', ( #67607 ), #42704, .T. ) ;
#125043=CARTESIAN_POINT ( 'NONE',  ( -11.64999999999999858, 12.50000000000000000, -5.802370205355746435 ) ) ;
#125044=DIRECTION ( 'NONE',  ( 0.000000000000000000, 0.000000000000000000, -1.000000000000000000 ) ) ;
#125045=DIRECTION ( 'NONE',  ( 0.000000000000000000, 0.000000000000000000, 1.000000000000000000 ) ) ;
#125046=EDGE_CURVE ( 'NONE', #98907, #22161, #44179, .T. ) ;
#125047=EDGE_LOOP ( 'NONE', ( #82526, #51393, #52678, #6912 ) ) ;
#125048=CIRCLE ( 'NONE', #49857, 0.06509327318403745899 ) ;
#125049=AXIS2_PLACEMENT_3D ( 'NONE', #41367, #81275, #19096 ) ;
#125050=DIRECTION ( 'NONE',  ( 0.000000000000000000, -0.9999939076577903929, 0.003490651415223739937 ) ) ;
#125051=ORIENTED_EDGE ( 'NONE', *, *, #30883, .F. ) ;
#125052=ADVANCED_FACE ( 'NONE', ( #21753 ), #82612, .T. ) ;
#125053=EDGE_CURVE ( 'NONE', #79044, #34557, #23675, .T. ) ;
#125054=ORIENTED_EDGE ( 'NONE', *, *, #29238, .T. ) ;
#125055=ORIENTED_EDGE ( 'NONE', *, *, #82389, .F. ) ;
#125056=EDGE_CURVE ( 'NONE', #107604, #62036, #1450, .T. ) ;
#125057=DIRECTION ( 'NONE',  ( -0.000000000000000000, -1.000000000000000000, -0.000000000000000000 ) ) ;
#125059=EDGE_CURVE ( 'NONE', #105966, #10113, #102863, .T. ) ;
#125060=FACE_BOUND ( 'NONE', #80489, .T. ) ;
#125061=CARTESIAN_POINT ( 'NONE',  ( -9.400000000000009237, 2.500000000000000000, -4.676537180435974328 ) ) ;
#125062=DIRECTION ( 'NONE',  ( 0.000000000000000000, -0.9999939076577903929, 0.003490651415223739937 ) ) ;
#125063=CARTESIAN_POINT ( 'NONE',  ( 11.44999999999990870, 2.500000000000000000, 6.841600689897072485 ) ) ;
#125064=VECTOR ( 'NONE', #81928, 1000.000000000000000 ) ;
#125065=EDGE_LOOP ( 'NONE', ( #96249, #89912 ) ) ;
#125066=DIRECTION ( 'NONE',  ( 0.000000000000000000, 0.000000000000000000, 1.000000000000000000 ) ) ;
#125067=DIRECTION ( 'NONE',  ( 0.000000000000000000, 0.000000000000000000, -1.000000000000000000 ) ) ;
#125068=EDGE_CURVE ( 'NONE', #11893, #28179, #6577, .T. ) ;
#125069=FACE_OUTER_BOUND ( 'NONE', #105379, .T. ) ;
#125070=CARTESIAN_POINT ( 'NONE',  ( -7.700000000000012612, 12.50000000000000000, 4.676537180435972552 ) ) ;
#125071=ORIENTED_EDGE ( 'NONE', *, *, #123327, .T. ) ;
#125073=AXIS2_PLACEMENT_3D ( 'NONE', #83811, #102798, #123721 ) ;
#125074=LINE ( 'NONE', #43312, #116401 ) ;
#125075=AXIS2_PLACEMENT_3D ( 'NONE', #21629, #101483, #42577 ) ;
#125076=VERTEX_POINT ( 'NONE', #2734 ) ;
#125077=DIRECTION ( 'NONE',  ( 0.000000000000000000, 0.000000000000000000, 1.000000000000000000 ) ) ;
#125078=ORIENTED_EDGE ( 'NONE', *, *, #109264, .T. ) ;
#125079=FACE_BOUND ( 'NONE', #65710, .T. ) ;
#125080=DIRECTION ( 'NONE',  ( -0.000000000000000000, -1.000000000000000000, -0.000000000000000000 ) ) ;
#125081=AXIS2_PLACEMENT_3D ( 'NONE', #50757, #41600, #14514 ) ;
#125082=CONICAL_SURFACE ( 'NONE', #68649, 0.1000000000000002554, 0.003490658503988666988 ) ;
#125083=ORIENTED_EDGE ( 'NONE', *, *, #46571, .T. ) ;
#125084=DIRECTION ( 'NONE',  ( 0.000000000000000000, 1.000000000000000000, 0.000000000000000000 ) ) ;
#125085=DIRECTION ( 'NONE',  ( 0.000000000000000000, 0.000000000000000000, 1.000000000000000000 ) ) ;
#125086=ORIENTED_EDGE ( 'NONE', *, *, #1637, .F. ) ;
#125087=ORIENTED_EDGE ( 'NONE', *, *, #4456, .T. ) ;
#125089=VERTEX_POINT ( 'NONE', #13190 ) ;
#125091=CARTESIAN_POINT ( 'NONE',  ( 8.949999999999915801, 2.500000000000000000, 6.841600689897072485 ) ) ;
#125092=CIRCLE ( 'NONE', #68661, 0.1000000000000002554 ) ;
#125093=DIRECTION ( 'NONE',  ( -0.000000000000000000, -1.000000000000000000, -0.000000000000000000 ) ) ;
#125094=DIRECTION ( 'NONE',  ( 0.000000000000000000, 1.000000000000000000, 0.000000000000000000 ) ) ;
#125095=FACE_OUTER_BOUND ( 'NONE', #6866, .T. ) ;
#125096=EDGE_CURVE ( 'NONE', #98747, #123356, #40077, .T. ) ;
#125097=FACE_OUTER_BOUND ( 'NONE', #83780, .T. ) ;
#125098=EDGE_CURVE ( 'NONE', #31027, #121877, #33512, .T. ) ;
#125099=CONICAL_SURFACE ( 'NONE', #51963, 0.1000000000000002554, 0.003490658503988666988 ) ;
#125100=VERTEX_POINT ( 'NONE', #71478 ) ;
#125101=EDGE_CURVE ( 'NONE', #25385, #3617, #58950, .T. ) ;
#125102=ORIENTED_EDGE ( 'NONE', *, *, #83433, .T. ) ;
#125103=PLANE ( 'NONE',  #103100 ) ;
#125104=CARTESIAN_POINT ( 'NONE',  ( 10.64999999999991331, 2.500000000000000000, 6.148780366869520897 ) ) ;
#125105=CIRCLE ( 'NONE', #39458, 0.06509327318403745899 ) ;
#125106=CARTESIAN_POINT ( 'NONE',  ( -12.89999999999999147, 12.50000000000000000, 5.022947341949748790 ) ) ;
#125107=VECTOR ( 'NONE', #28932, 1000.000000000000000 ) ;
#125108=CARTESIAN_POINT ( 'NONE',  ( -4.600000000000025402, 2.500000000000000000, 4.330127018922196314 ) ) ;
#125109=ORIENTED_EDGE ( 'NONE', *, *, #21427, .T. ) ;
#125110=EDGE_LOOP ( 'NONE', ( #35089, #124442, #113840, #100447 ) ) ;
#125111=FACE_BOUND ( 'NONE', #66914, .T. ) ;
#125112=EDGE_LOOP ( 'NONE', ( #25049, #54528 ) ) ;
#125113=EDGE_CURVE ( 'NONE', #94097, #9132, #430, .T. ) ;
#125114=CARTESIAN_POINT ( 'NONE',  ( 11.64999999999990621, 2.500000000000000000, -2.165063509461101710 ) ) ;
#125115=CARTESIAN_POINT ( 'NONE',  ( -7.050000000000016698, 12.50000000000000000, -6.495190528383302464 ) ) ;
#125116=ADVANCED_FACE ( 'NONE', ( #12552 ), #71450, .T. ) ;
#125117=ORIENTED_EDGE ( 'NONE', *, *, #79108, .T. ) ;
#125118=FACE_OUTER_BOUND ( 'NONE', #129435, .T. ) ;
#125119=AXIS2_PLACEMENT_3D ( 'NONE', #24726, #45018, #113098 ) ;
#125120=DIRECTION ( 'NONE',  ( -0.000000000000000000, -1.000000000000000000, -0.000000000000000000 ) ) ;
#125121=ADVANCED_FACE ( 'NONE', ( #810 ), #10793, .T. ) ;
#125122=DIRECTION ( 'NONE',  ( -4.274815082592931898E-19, -0.9999939076577903929, -0.003490651415223739937 ) ) ;
#125123=EDGE_CURVE ( 'NONE', #35030, #106850, #8751, .T. ) ;
#125124=CARTESIAN_POINT ( 'NONE',  ( 6.899999999999928413, 2.500000000000000000, 4.676537180435972552 ) ) ;
#125125=DIRECTION ( 'NONE',  ( 0.000000000000000000, 0.000000000000000000, 1.000000000000000000 ) ) ;
#125126=CARTESIAN_POINT ( 'NONE',  ( -4.150000000000028777, 2.500000000000000000, -5.902370205355750521 ) ) ;
#125127=DIRECTION ( 'NONE',  ( -0.000000000000000000, -1.000000000000000000, -0.000000000000000000 ) ) ;
#125128=DIRECTION ( 'NONE',  ( -0.000000000000000000, 1.000000000000000000, -0.000000000000000000 ) ) ;
#125129=AXIS2_PLACEMENT_3D ( 'NONE', #56863, #64764, #64126 ) ;
#125130=DIRECTION ( 'NONE',  ( 0.000000000000000000, 0.000000000000000000, -1.000000000000000000 ) ) ;
#125131=ADVANCED_FACE ( 'NONE', ( #100933 ), #51224, .T. ) ;
#125132=AXIS2_PLACEMENT_3D ( 'NONE', #13792, #35392, #113291 ) ;
#125133=ORIENTED_EDGE ( 'NONE', *, *, #205, .F. ) ;
#125134=VERTEX_POINT ( 'NONE', #91129 ) ;
#125135=CARTESIAN_POINT ( 'NONE',  ( 6.849999999999930367, 2.500000000000000000, -6.841600689897078702 ) ) ;
#125136=ORIENTED_EDGE ( 'NONE', *, *, #10650, .T. ) ;
#125137=FACE_OUTER_BOUND ( 'NONE', #20631, .T. ) ;
#125138=VERTEX_POINT ( 'NONE', #22409 ) ;
#125139=VERTEX_POINT ( 'NONE', #30938 ) ;
#125140=ORIENTED_EDGE ( 'NONE', *, *, #47535, .F. ) ;
#125141=AXIS2_PLACEMENT_3D ( 'NONE', #115933, #55724, #76659 ) ;
#125142=DIRECTION ( 'NONE',  ( 0.000000000000000000, 1.000000000000000000, 0.000000000000000000 ) ) ;
#125143=CARTESIAN_POINT ( 'NONE',  ( 3.749999999999944045, 2.500000000000000000, -7.288010851410854585 ) ) ;
#125144=CIRCLE ( 'NONE', #85424, 0.1000000000000002554 ) ;
#125145=CARTESIAN_POINT ( 'NONE',  ( 65.39894234709436205, -3.129862333804463326, -5.811320850207112088 ) ) ;
#125146=DIRECTION ( 'NONE',  ( 0.000000000000000000, 0.000000000000000000, 1.000000000000000000 ) ) ;
#125147=LINE ( 'NONE', #16457, #1567 ) ;
#125148=AXIS2_PLACEMENT_3D ( 'NONE', #111735, #22085, #4328 ) ;
#125149=EDGE_CURVE ( 'NONE', #16388, #114720, #53146, .T. ) ;
#125150=ORIENTED_EDGE ( 'NONE', *, *, #39793, .F. ) ;
#125151=CARTESIAN_POINT ( 'NONE',  ( 0.8499999999999536815, 2.500000000000000000, 6.495190528383297135 ) ) ;
#125152=VERTEX_POINT ( 'NONE', #95639 ) ;
#125153=AXIS2_PLACEMENT_3D ( 'NONE', #72945, #123332, #52647 ) ;
#125154=AXIS2_PLACEMENT_3D ( 'NONE', #96066, #78384, #126177 ) ;
#125155=ORIENTED_EDGE ( 'NONE', *, *, #19982, .F. ) ;
#125156=EDGE_LOOP ( 'NONE', ( #118681, #60975, #61053, #114182 ) ) ;
#125157=CARTESIAN_POINT ( 'NONE',  ( -7.100000000000018296, 2.500000000000000000, -4.230127018922201998 ) ) ;
#125158=ORIENTED_EDGE ( 'NONE', *, *, #73106, .F. ) ;
#125159=VERTEX_POINT ( 'NONE', #4022 ) ;
#125160=ORIENTED_EDGE ( 'NONE', *, *, #82509, .T. ) ;
#125161=DIRECTION ( 'NONE',  ( 0.000000000000000000, 0.000000000000000000, 1.000000000000000000 ) ) ;
#125162=DIRECTION ( 'NONE',  ( -0.000000000000000000, -1.000000000000000000, -0.000000000000000000 ) ) ;
#125163=CARTESIAN_POINT ( 'NONE',  ( 11.64999999999990621, 2.500000000000000000, 6.495190528383297135 ) ) ;
#125164=ADVANCED_FACE ( 'NONE', ( #124459 ), #52686, .T. ) ;
#125165=CARTESIAN_POINT ( 'NONE',  ( -13.34999999999999076, 2.500000000000000000, -2.857883832488651521 ) ) ;
#125166=CARTESIAN_POINT ( 'NONE',  ( -12.09999999999999609, 12.50000000000000000, -5.088040615133788691 ) ) ;
#125167=CARTESIAN_POINT ( 'NONE',  ( 13.74999999999989342, 2.500000000000000000, -1.472243186433550122 ) ) ;
#125168=AXIS2_PLACEMENT_3D ( 'NONE', #124297, #113837, #34650 ) ;
#125169=ORIENTED_EDGE ( 'NONE', *, *, #97444, .T. ) ;
#125170=CARTESIAN_POINT ( 'NONE',  ( 15.39999999999989200, 2.500000000000000000, -0.6928203230275542523 ) ) ;
#125171=ORIENTED_EDGE ( 'NONE', *, *, #60662, .T. ) ;
#125172=VECTOR ( 'NONE', #122953, 1000.000000000000000 ) ;
#125173=PLANE ( 'NONE',  #77762 ) ;
#125174=VECTOR ( 'NONE', #19224, 1000.000000000000000 ) ;
#125175=EDGE_LOOP ( 'NONE', ( #78759, #671 ) ) ;
#125177=CIRCLE ( 'NONE', #102193, 0.06509327318403745899 ) ;
#125178=VERTEX_POINT ( 'NONE', #56345 ) ;
#125179=EDGE_CURVE ( 'NONE', #126922, #56443, #104897, .T. ) ;
#125180=VERTEX_POINT ( 'NONE', #5946 ) ;
#125181=DIRECTION ( 'NONE',  ( 0.000000000000000000, 1.000000000000000000, 0.000000000000000000 ) ) ;
#125182=DIRECTION ( 'NONE',  ( -0.000000000000000000, 1.000000000000000000, -0.000000000000000000 ) ) ;
#125183=AXIS2_PLACEMENT_3D ( 'NONE', #94889, #5842, #45799 ) ;
#125184=AXIS2_PLACEMENT_3D ( 'NONE', #18088, #17431, #117553 ) ;
#125185=CARTESIAN_POINT ( 'NONE',  ( -14.99999999999994671, 12.50000000000000000, -0.06509327318403743123 ) ) ;
#125186=DIRECTION ( 'NONE',  ( -0.000000000000000000, -1.000000000000000000, -0.000000000000000000 ) ) ;
#125187=DIRECTION ( 'NONE',  ( 0.000000000000000000, 1.000000000000000000, 0.000000000000000000 ) ) ;
#125188=ORIENTED_EDGE ( 'NONE', *, *, #74151, .F. ) ;
#125189=LINE ( 'NONE', #43429, #26822 ) ;
#125190=CARTESIAN_POINT ( 'NONE',  ( 11.89999999999990798, 2.500000000000000000, 4.676537180435972552 ) ) ;
#125191=DIRECTION ( 'NONE',  ( 0.000000000000000000, -0.9999939076577903929, 0.003490651415223739937 ) ) ;
#125192=DIRECTION ( 'NONE',  ( 0.000000000000000000, 0.000000000000000000, 1.000000000000000000 ) ) ;
#125193=CIRCLE ( 'NONE', #41591, 0.06509327318403745899 ) ;
#125194=FACE_OUTER_BOUND ( 'NONE', #99060, .T. ) ;
#125195=AXIS2_PLACEMENT_3D ( 'NONE', #11688, #11031, #52913 ) ;
#125196=VERTEX_POINT ( 'NONE', #85169 ) ;
#125197=VERTEX_POINT ( 'NONE', #64241 ) ;
#125198=ORIENTED_EDGE ( 'NONE', *, *, #3346, .T. ) ;
#125199=DIRECTION ( 'NONE',  ( 0.000000000000000000, 0.000000000000000000, -1.000000000000000000 ) ) ;
#125200=DIRECTION ( 'NONE',  ( -0.000000000000000000, 1.000000000000000000, -0.000000000000000000 ) ) ;
#125201=CONICAL_SURFACE ( 'NONE', #12321, 0.1000000000000000472, 0.003490658503988666988 ) ;
#125202=EDGE_CURVE ( 'NONE', #120397, #25624, #90312, .T. ) ;
#125203=CIRCLE ( 'NONE', #93813, 0.09999999999999999167 ) ;
#125205=CARTESIAN_POINT ( 'NONE',  ( -11.89999999999999680, 2.500000000000000000, -4.776537180435975749 ) ) ;
#125206=LINE ( 'NONE', #27011, #115603 ) ;
#125207=CARTESIAN_POINT ( 'NONE',  ( 5.199999999999935341, 2.500000000000000000, -4.083716857408426826 ) ) ;
#125208=DIRECTION ( 'NONE',  ( 0.000000000000000000, -0.9999939076577903929, 0.003490651415223739937 ) ) ;
#125209=ORIENTED_EDGE ( 'NONE', *, *, #3910, .T. ) ;
#125210=DIRECTION ( 'NONE',  ( 0.000000000000000000, 0.000000000000000000, -1.000000000000000000 ) ) ;
#125211=DIRECTION ( 'NONE',  ( 0.000000000000000000, 0.000000000000000000, 1.000000000000000000 ) ) ;
#125212=AXIS2_PLACEMENT_3D ( 'NONE', #12785, #92011, #2318 ) ;
#125213=ORIENTED_EDGE ( 'NONE', *, *, #25813, .T. ) ;
#125214=ADVANCED_FACE ( 'NONE', ( #46524 ), #34807, .T. ) ;
#125215=ADVANCED_FACE ( 'NONE', ( #45901 ), #125830, .T. ) ;
#125216=EDGE_CURVE ( 'NONE', #61323, #7453, #48477, .T. ) ;
#125217=DIRECTION ( 'NONE',  ( -0.000000000000000000, 1.000000000000000000, -0.000000000000000000 ) ) ;
#125218=ADVANCED_FACE ( 'NONE', ( #75992 ), #111152, .T. ) ;
#125219=AXIS2_PLACEMENT_3D ( 'NONE', #99733, #69610, #91191 ) ;
#125220=CARTESIAN_POINT ( 'NONE',  ( -8.550000000000009592, 12.50000000000000000, 6.906693963081109722 ) ) ;
#125221=CARTESIAN_POINT ( 'NONE',  ( 6.249999999999932498, 2.500000000000000000, -2.857883832488653741 ) ) ;
#125222=ORIENTED_EDGE ( 'NONE', *, *, #112984, .F. ) ;
#125223=DIRECTION ( 'NONE',  ( -0.000000000000000000, 1.000000000000000000, -0.000000000000000000 ) ) ;
#125224=ORIENTED_EDGE ( 'NONE', *, *, #100392, .T. ) ;
#125225=DIRECTION ( 'NONE',  ( 0.000000000000000000, 1.000000000000000000, 0.000000000000000000 ) ) ;
#125226=CIRCLE ( 'NONE', #112710, 0.1000000000000002554 ) ;
#125227=CARTESIAN_POINT ( 'NONE',  ( 11.84999999999990372, 2.500000000000000000, 2.411473670974873862 ) ) ;
#125228=ADVANCED_FACE ( 'NONE', ( #113996 ), #33908, .T. ) ;
#125229=EDGE_LOOP ( 'NONE', ( #107325, #37043 ) ) ;
#125230=ADVANCED_FACE ( 'NONE', ( #125097 ), #73602, .T. ) ;
#125232=EDGE_CURVE ( 'NONE', #44668, #73184, #66801, .T. ) ;
#125233=AXIS2_PLACEMENT_3D ( 'NONE', #22971, #31498, #92336 ) ;
#125234=CIRCLE ( 'NONE', #12352, 0.06509327318403745899 ) ;
#125235=DIRECTION ( 'NONE',  ( 0.000000000000000000, 0.000000000000000000, -1.000000000000000000 ) ) ;
#125236=CIRCLE ( 'NONE', #112720, 0.06509327318403743123 ) ;
#125238=DIRECTION ( 'NONE',  ( 0.000000000000000000, 0.000000000000000000, 1.000000000000000000 ) ) ;
#125239=AXIS2_PLACEMENT_3D ( 'NONE', #12310, #51612, #101353 ) ;
#125240=AXIS2_PLACEMENT_3D ( 'NONE', #124085, #74343, #114264 ) ;
#125241=ORIENTED_EDGE ( 'NONE', *, *, #26353, .F. ) ;
#125242=VERTEX_POINT ( 'NONE', #75342 ) ;
#125243=DIRECTION ( 'NONE',  ( 0.000000000000000000, 0.000000000000000000, 1.000000000000000000 ) ) ;
#125244=DIRECTION ( 'NONE',  ( 0.000000000000000000, 0.000000000000000000, 1.000000000000000000 ) ) ;
#125245=EDGE_LOOP ( 'NONE', ( #59864, #95228 ) ) ;
#125246=LINE ( 'NONE', #113482, #113696 ) ;
#125247=DIRECTION ( 'NONE',  ( 0.000000000000000000, 0.000000000000000000, 1.000000000000000000 ) ) ;
#125248=EDGE_LOOP ( 'NONE', ( #59140, #51582, #30346, #97137 ) ) ;
#125249=CARTESIAN_POINT ( 'NONE',  ( -3.150000000000029221, 2.500000000000000000, 2.511473670974873507 ) ) ;
#125250=CARTESIAN_POINT ( 'NONE',  ( -10.00000000000000355, 2.500000000000000000, 3.637306695894644726 ) ) ;
#125251=DIRECTION ( 'NONE',  ( -0.000000000000000000, -1.000000000000000000, -0.000000000000000000 ) ) ;
#125252=AXIS2_PLACEMENT_3D ( 'NONE', #87897, #19836, #10006 ) ;
#125253=CARTESIAN_POINT ( 'NONE',  ( 10.84999999999991260, 2.500000000000000000, -2.265063509461101798 ) ) ;
#125254=CARTESIAN_POINT ( 'NONE',  ( -13.74999999999995381, 2.500000000000000000, -2.265063509461099578 ) ) ;
#125255=DIRECTION ( 'NONE',  ( 0.000000000000000000, 0.000000000000000000, -1.000000000000000000 ) ) ;
#125256=CONICAL_SURFACE ( 'NONE', #121050, 0.1000000000000002554, 0.003490658503988666988 ) ;
#125257=CONICAL_SURFACE ( 'NONE', #3972, 0.09999999999999982514, 0.003490658503988666988 ) ;
#125258=ORIENTED_EDGE ( 'NONE', *, *, #91626, .T. ) ;
#125259=ORIENTED_EDGE ( 'NONE', *, *, #94771, .T. ) ;
#125260=ORIENTED_EDGE ( 'NONE', *, *, #7895, .F. ) ;
#125261=EDGE_LOOP ( 'NONE', ( #98105, #63531 ) ) ;
#125262=CARTESIAN_POINT ( 'NONE',  ( 4.199999999999939782, 2.500000000000000000, -2.276824562219559311E-15 ) ) ;
#125263=CARTESIAN_POINT ( 'NONE',  ( -3.750000000000031086, 12.50000000000000000, -5.802370205355749988 ) ) ;
#125264=LINE ( 'NONE', #84035, #76123 ) ;
#125265=ORIENTED_EDGE ( 'NONE', *, *, #41155, .T. ) ;
#125266=FACE_BOUND ( 'NONE', #71485, .T. ) ;
#125267=DIRECTION ( 'NONE',  ( 0.000000000000000000, 0.000000000000000000, -1.000000000000000000 ) ) ;
#125268=PLANE ( 'NONE',  #73098 ) ;
#125269=AXIS2_PLACEMENT_3D ( 'NONE', #47932, #95089, #17799 ) ;
#125270=CIRCLE ( 'NONE', #85555, 0.06509327318403745899 ) ;
#125271=EDGE_CURVE ( 'NONE', #53553, #43500, #98632, .T. ) ;
#125272=CARTESIAN_POINT ( 'NONE',  ( -1.450000000000035483, 12.50000000000000000, 1.818653347947321475 ) ) ;
#125273=AXIS2_PLACEMENT_3D ( 'NONE', #115282, #117218, #34848 ) ;
#125274=DIRECTION ( 'NONE',  ( 0.000000000000000000, 1.000000000000000000, 0.000000000000000000 ) ) ;
#125275=ADVANCED_FACE ( 'NONE', ( #93705 ), #107046, .T. ) ;
#125277=DIRECTION ( 'NONE',  ( -4.274815082592931898E-19, -0.9999939076577903929, -0.003490651415223739937 ) ) ;
#125278=CARTESIAN_POINT ( 'NONE',  ( -11.84999999999999787, 2.500000000000000000, -2.411473670974874306 ) ) ;
#125279=DIRECTION ( 'NONE',  ( -0.000000000000000000, -1.000000000000000000, -0.000000000000000000 ) ) ;
#125280=DIRECTION ( 'NONE',  ( -0.000000000000000000, 1.000000000000000000, -0.000000000000000000 ) ) ;
#125281=VECTOR ( 'NONE', #40911, 1000.000000000000000 ) ;
#125282=CARTESIAN_POINT ( 'NONE',  ( 12.69999999999989981, 2.500000000000000000, -0.3464101615137783474 ) ) ;
#125283=EDGE_CURVE ( 'NONE', #64666, #62380, #83873, .T. ) ;
#125284=CIRCLE ( 'NONE', #68844, 0.09999999999999982514 ) ;
#125285=ORIENTED_EDGE ( 'NONE', *, *, #128561, .T. ) ;
#125286=ORIENTED_EDGE ( 'NONE', *, *, #34112, .F. ) ;
#125287=CONICAL_SURFACE ( 'NONE', #18759, 0.1000000000000002554, 0.003490658503988666988 ) ;
#125288=ORIENTED_EDGE ( 'NONE', *, *, #63931, .T. ) ;
#125289=VERTEX_POINT ( 'NONE', #6573 ) ;
#125290=DIRECTION ( 'NONE',  ( -0.000000000000000000, -1.000000000000000000, -0.000000000000000000 ) ) ;
#125291=ORIENTED_EDGE ( 'NONE', *, *, #38288, .T. ) ;
#125292=DIRECTION ( 'NONE',  ( -0.000000000000000000, -1.000000000000000000, -0.000000000000000000 ) ) ;
#125293=VERTEX_POINT ( 'NONE', #114623 ) ;
#125294=ORIENTED_EDGE ( 'NONE', *, *, #49847, .F. ) ;
#125295=DIRECTION ( 'NONE',  ( 0.000000000000000000, 0.000000000000000000, 1.000000000000000000 ) ) ;
#125296=CARTESIAN_POINT ( 'NONE',  ( 9.112263991835156673, -1.499999999999809042, 9.392448311626335311 ) ) ;
#125297=DIRECTION ( 'NONE',  ( 0.000000000000000000, 1.000000000000000000, 0.000000000000000000 ) ) ;
#125298=DIRECTION ( 'NONE',  ( 0.000000000000000000, 0.000000000000000000, 1.000000000000000000 ) ) ;
#125299=AXIS2_PLACEMENT_3D ( 'NONE', #107144, #17469, #56112 ) ;
#125300=LINE ( 'NONE', #66371, #120832 ) ;
#125301=VERTEX_POINT ( 'NONE', #115240 ) ;
#125302=EDGE_LOOP ( 'NONE', ( #124013, #64275 ) ) ;
#125303=ORIENTED_EDGE ( 'NONE', *, *, #116245, .F. ) ;
#125304=CARTESIAN_POINT ( 'NONE',  ( -1.850000000000033396, 12.50000000000000000, -6.148780366869526226 ) ) ;
#125305=ORIENTED_EDGE ( 'NONE', *, *, #89146, .F. ) ;
#125306=CARTESIAN_POINT ( 'NONE',  ( -11.24999999999999822, 12.50000000000000000, 5.867463478539781896 ) ) ;
#125307=VERTEX_POINT ( 'NONE', #123790 ) ;
#125308=ORIENTED_EDGE ( 'NONE', *, *, #8309, .T. ) ;
#125309=CIRCLE ( 'NONE', #114829, 0.06509327318403745899 ) ;
#125310=CARTESIAN_POINT ( 'NONE',  ( 15.59999999999988951, 2.500000000000000000, -0.2464101615137783419 ) ) ;
#125311=DIRECTION ( 'NONE',  ( -4.274815082592931898E-19, -0.9999939076577903929, -0.003490651415223739937 ) ) ;
#125312=CARTESIAN_POINT ( 'NONE',  ( -2.700000000000030820, 2.500000000000000000, 0.2464101615137735679 ) ) ;
#125314=CARTESIAN_POINT ( 'NONE',  ( 6.899999999999928413, 12.50000000000000000, 4.048810130592458201 ) ) ;
#125315=DIRECTION ( 'NONE',  ( 0.000000000000000000, -0.000000000000000000, 1.000000000000000000 ) ) ;
#125316=PLANE ( 'NONE',  #39352 ) ;
#125317=CIRCLE ( 'NONE', #127381, 0.1000000000000000472 ) ;
#125318=VERTEX_POINT ( 'NONE', #45258 ) ;
#125319=CARTESIAN_POINT ( 'NONE',  ( -8.550000000000014921, 12.50000000000000000, -6.083687093685483660 ) ) ;
#125320=ORIENTED_EDGE ( 'NONE', *, *, #37320, .T. ) ;
#125321=DIRECTION ( 'NONE',  ( -0.000000000000000000, -1.000000000000000000, -0.000000000000000000 ) ) ;
#125322=AXIS2_PLACEMENT_3D ( 'NONE', #43907, #82542, #3324 ) ;
#125323=AXIS2_PLACEMENT_3D ( 'NONE', #59421, #99327, #9650 ) ;
#125324=ORIENTED_EDGE ( 'NONE', *, *, #1494, .F. ) ;
#125325=FACE_OUTER_BOUND ( 'NONE', #72234, .T. ) ;
#125326=FACE_OUTER_BOUND ( 'NONE', #29386, .T. ) ;
#125327=EDGE_CURVE ( 'NONE', #22783, #22326, #42234, .T. ) ;
#125328=ORIENTED_EDGE ( 'NONE', *, *, #122085, .T. ) ;
#125329=CIRCLE ( 'NONE', #71045, 0.06509327318403745899 ) ;
#125330=FACE_OUTER_BOUND ( 'NONE', #32430, .T. ) ;
#125331=ADVANCED_FACE ( 'NONE', ( #108027 ), #12954, .T. ) ;
#125332=DIRECTION ( 'NONE',  ( -0.000000000000000000, 1.000000000000000000, -0.000000000000000000 ) ) ;
#125333=ORIENTED_EDGE ( 'NONE', *, *, #53147, .T. ) ;
#125334=LINE ( 'NONE', #105702, #21435 ) ;
#125335=VECTOR ( 'NONE', #111492, 1000.000000000000000 ) ;
#125336=CIRCLE ( 'NONE', #85615, 0.1000000000000002554 ) ;
#125337=LINE ( 'NONE', #16008, #96787 ) ;
#125338=EDGE_LOOP ( 'NONE', ( #54858, #49426, #42813, #63332 ) ) ;
#125339=EDGE_CURVE ( 'NONE', #127915, #87106, #102840, .T. ) ;
#125340=VERTEX_POINT ( 'NONE', #79863 ) ;
#125341=CARTESIAN_POINT ( 'NONE',  ( 0.8499999999999545697, 2.500000000000000000, 2.857883832488649301 ) ) ;
#125342=DIRECTION ( 'NONE',  ( 0.000000000000000000, 0.000000000000000000, -1.000000000000000000 ) ) ;
#125344=DIRECTION ( 'NONE',  ( 0.000000000000000000, 0.000000000000000000, 1.000000000000000000 ) ) ;
#125345=DIRECTION ( 'NONE',  ( 0.000000000000000000, -0.9999939076577903929, 0.003490651415223739937 ) ) ;
#125346=DIRECTION ( 'NONE',  ( 0.000000000000000000, 0.000000000000000000, 1.000000000000000000 ) ) ;
#125347=AXIS2_PLACEMENT_3D ( 'NONE', #87261, #9362, #39496 ) ;
#125348=ORIENTED_EDGE ( 'NONE', *, *, #128595, .T. ) ;
#125349=DIRECTION ( 'NONE',  ( 0.000000000000000000, 1.000000000000000000, 0.000000000000000000 ) ) ;
#125350=VECTOR ( 'NONE', #90356, 1000.000000000000000 ) ;
#125352=ORIENTED_EDGE ( 'NONE', *, *, #35722, .T. ) ;
#125353=DIRECTION ( 'NONE',  ( -4.274815082592931898E-19, -0.9999939076577903929, -0.003490651415223739937 ) ) ;
#125355=CARTESIAN_POINT ( 'NONE',  ( -12.09999999999999609, 2.500000000000000000, 4.330127018922196314 ) ) ;
#125356=AXIS2_PLACEMENT_3D ( 'NONE', #42123, #61777, #72871 ) ;
#125357=VERTEX_POINT ( 'NONE', #69391 ) ;
#125358=CIRCLE ( 'NONE', #45955, 0.06509327318403745899 ) ;
#125359=CIRCLE ( 'NONE', #41758, 0.1000000000000002554 ) ;
#125360=ADVANCED_FACE ( 'NONE', ( #98850 ), #10887, .T. ) ;
#125361=CARTESIAN_POINT ( 'NONE',  ( -10.20000000000000284, 2.500000000000000000, 3.883716857408421319 ) ) ;
#125362=CARTESIAN_POINT ( 'NONE',  ( -11.84999999999999609, 2.500000000000000000, 1.718653347947321386 ) ) ;
#125363=EDGE_CURVE ( 'NONE', #108419, #7922, #96575, .T. ) ;
#125364=ADVANCED_FACE ( 'NONE', ( #117176 ), #98205, .T. ) ;
#125365=EDGE_CURVE ( 'NONE', #126837, #36298, #40179, .T. ) ;
#125366=AXIS2_PLACEMENT_3D ( 'NONE', #94320, #4636, #44595 ) ;
#125367=EDGE_CURVE ( 'NONE', #43127, #105608, #117405, .T. ) ;
#125368=ORIENTED_EDGE ( 'NONE', *, *, #13888, .T. ) ;
#125369=CARTESIAN_POINT ( 'NONE',  ( -0.4000000000000404898, 12.50000000000000000, 5.088040615133786027 ) ) ;
#125370=AXIS2_PLACEMENT_3D ( 'NONE', #14580, #92507, #32974 ) ;
#125371=AXIS2_PLACEMENT_3D ( 'NONE', #4617, #45227, #53747 ) ;
#125373=VERTEX_POINT ( 'NONE', #8524 ) ;
#125374=FACE_OUTER_BOUND ( 'NONE', #4871, .T. ) ;
#125375=ADVANCED_FACE ( 'NONE', ( #127669 ), #77283, .T. ) ;
#125376=ADVANCED_FACE ( 'NONE', ( #89044 ), #13038, .T. ) ;
#125377=EDGE_LOOP ( 'NONE', ( #19357, #109610, #28648, #17344 ) ) ;
#125378=DIRECTION ( 'NONE',  ( 0.000000000000000000, -0.000000000000000000, 1.000000000000000000 ) ) ;
#125379=DIRECTION ( 'NONE',  ( -4.274815082592931898E-19, -0.9999939076577903929, -0.003490651415223739937 ) ) ;
#125381=DIRECTION ( 'NONE',  ( -0.000000000000000000, 1.000000000000000000, -0.000000000000000000 ) ) ;
#125382=ORIENTED_EDGE ( 'NONE', *, *, #33167, .F. ) ;
#125383=ADVANCED_FACE ( 'NONE', ( #27519 ), #77921, .T. ) ;
#125384=FACE_BOUND ( 'NONE', #63845, .T. ) ;
#125385=ADVANCED_FACE ( 'NONE', ( #78598 ), #119143, .T. ) ;
#125386=CARTESIAN_POINT ( 'NONE',  ( -2.300000000000033573, 2.500000000000000000, 4.676537180435972552 ) ) ;
#125387=ORIENTED_EDGE ( 'NONE', *, *, #58610, .T. ) ;
#125388=AXIS2_PLACEMENT_3D ( 'NONE', #121919, #91812, #44651 ) ;
#125390=ADVANCED_FACE ( 'NONE', ( #28842 ), #68750, .T. ) ;
#125391=DIRECTION ( 'NONE',  ( 0.000000000000000000, 0.000000000000000000, -1.000000000000000000 ) ) ;
#125393=ORIENTED_EDGE ( 'NONE', *, *, #87935, .T. ) ;
#125394=ORIENTED_EDGE ( 'NONE', *, *, #12606, .F. ) ;
#125395=ORIENTED_EDGE ( 'NONE', *, *, #66681, .T. ) ;
#125396=CARTESIAN_POINT ( 'NONE',  ( -8.550000000000011369, 2.500000000000000000, 1.818653347947321475 ) ) ;
#125397=CARTESIAN_POINT ( 'NONE',  ( 3.677269697638545054, 2.500000000000000000, 8.999999999909123360 ) ) ;
#125398=CARTESIAN_POINT ( 'NONE',  ( -4.200000000000025935, 12.50000000000000000, -2.385244779468109755E-15 ) ) ;
#125399=FACE_BOUND ( 'NONE', #13106, .T. ) ;
#125400=ORIENTED_EDGE ( 'NONE', *, *, #58616, .T. ) ;
#125402=DIRECTION ( 'NONE',  ( 0.000000000000000000, 1.000000000000000000, 0.000000000000000000 ) ) ;
#125403=CARTESIAN_POINT ( 'NONE',  ( -1.050000000000037348, 2.500000000000000000, -6.841600689897078702 ) ) ;
#125404=DIRECTION ( 'NONE',  ( 0.000000000000000000, 0.000000000000000000, 1.000000000000000000 ) ) ;
#125405=DIRECTION ( 'NONE',  ( 0.000000000000000000, 1.000000000000000000, 0.000000000000000000 ) ) ;
#125407=AXIS2_PLACEMENT_3D ( 'NONE', #24844, #26140, #6450 ) ;
#125408=DIRECTION ( 'NONE',  ( 0.000000000000000000, 1.000000000000000000, 0.000000000000000000 ) ) ;
#125409=DIRECTION ( 'NONE',  ( 0.000000000000000000, 0.000000000000000000, 1.000000000000000000 ) ) ;
#125410=CARTESIAN_POINT ( 'NONE',  ( -6.050000000000018474, 2.500000000000000000, 2.411473670974873862 ) ) ;
#125411=CONICAL_SURFACE ( 'NONE', #12530, 0.1000000000000002554, 0.003490658503988666988 ) ;
#125412=VERTEX_POINT ( 'NONE', #10469 ) ;
#125413=ORIENTED_EDGE ( 'NONE', *, *, #105605, .F. ) ;
#125414=ORIENTED_EDGE ( 'NONE', *, *, #8200, .T. ) ;
#125415=EDGE_LOOP ( 'NONE', ( #125772, #33862 ) ) ;
#125417=CARTESIAN_POINT ( 'NONE',  ( 1.899999999999949507, 12.50000000000000000, 4.611443907251934426 ) ) ;
#125418=FACE_OUTER_BOUND ( 'NONE', #112029, .T. ) ;
#125419=VERTEX_POINT ( 'NONE', #70050 ) ;
#125420=FACE_BOUND ( 'NONE', #87042, .T. ) ;
#125421=CARTESIAN_POINT ( 'NONE',  ( -14.54999999999998472, 2.500000000000000000, 2.165063509461101265 ) ) ;
#125422=VECTOR ( 'NONE', #22501, 1000.000000000000000 ) ;
#125423=AXIS2_PLACEMENT_3D ( 'NONE', #16368, #96880, #56310 ) ;
#125424=EDGE_CURVE ( 'NONE', #27855, #50402, #30785, .T. ) ;
#125425=DIRECTION ( 'NONE',  ( -0.000000000000000000, -1.000000000000000000, -0.000000000000000000 ) ) ;
#125426=EDGE_CURVE ( 'NONE', #81351, #90210, #52768, .T. ) ;
#125427=ORIENTED_EDGE ( 'NONE', *, *, #52420, .T. ) ;
#125428=CARTESIAN_POINT ( 'NONE',  ( 4.999999999999933387, 2.500000000000000000, 5.122947341949749323 ) ) ;
#125429=FACE_OUTER_BOUND ( 'NONE', #58518, .T. ) ;
#125430=DIRECTION ( 'NONE',  ( -0.000000000000000000, -1.000000000000000000, -0.000000000000000000 ) ) ;
#125431=EDGE_LOOP ( 'NONE', ( #44597, #82363 ) ) ;
#125432=DIRECTION ( 'NONE',  ( 0.000000000000000000, 0.000000000000000000, 1.000000000000000000 ) ) ;
#125433=VERTEX_POINT ( 'NONE', #81160 ) ;
#125434=VERTEX_POINT ( 'NONE', #20944 ) ;
#125435=EDGE_LOOP ( 'NONE', ( #42145, #115299 ) ) ;
#125436=CARTESIAN_POINT ( 'NONE',  ( -2.100000000000033396, 2.500000000000000000, -3.537306695894649966 ) ) ;
#125437=CARTESIAN_POINT ( 'NONE',  ( -5.000000000000023093, 2.500000000000000000, 0.7928203230275495672 ) ) ;
#125438=CARTESIAN_POINT ( 'NONE',  ( 1.899999999999951283, 2.500000000000000000, -4.676537180435977881 ) ) ;
#125439=ORIENTED_EDGE ( 'NONE', *, *, #7098, .F. ) ;
#125440=DIRECTION ( 'NONE',  ( 0.000000000000000000, 0.000000000000000000, 1.000000000000000000 ) ) ;
#125441=PLANE ( 'NONE',  #5206 ) ;
#125442=AXIS2_PLACEMENT_3D ( 'NONE', #125282, #114804, #25784 ) ;
#125443=DIRECTION ( 'NONE',  ( 0.000000000000000000, -0.9999939076577903929, 0.003490651415223739937 ) ) ;
#125445=DIRECTION ( 'NONE',  ( 0.000000000000000000, 0.000000000000000000, -1.000000000000000000 ) ) ;
#125446=CARTESIAN_POINT ( 'NONE',  ( -12.49999999999999289, 12.50000000000000000, -0.6928203230275500335 ) ) ;
#125447=ORIENTED_EDGE ( 'NONE', *, *, #86523, .F. ) ;
#125448=CARTESIAN_POINT ( 'NONE',  ( 15.79999999999989058, 2.500000000000000000, -2.385244779468109755E-15 ) ) ;
#125449=AXIS2_PLACEMENT_3D ( 'NONE', #63399, #94789, #93503 ) ;
#125450=VERTEX_POINT ( 'NONE', #20302 ) ;
#125451=ORIENTED_EDGE ( 'NONE', *, *, #117460, .T. ) ;
#125452=CARTESIAN_POINT ( 'NONE',  ( 13.74999999999989875, 2.500000000000000000, 1.572243186433545548 ) ) ;
#125453=CARTESIAN_POINT ( 'NONE',  ( 12.04999999999990479, 12.50000000000000000, 2.165063509461097713 ) ) ;
#125454=FACE_OUTER_BOUND ( 'NONE', #64925, .T. ) ;
#125455=AXIS2_PLACEMENT_3D ( 'NONE', #115902, #15760, #19474 ) ;
#125456=ORIENTED_EDGE ( 'NONE', *, *, #70579, .F. ) ;
#125457=ORIENTED_EDGE ( 'NONE', *, *, #32754, .T. ) ;
#125458=AXIS2_PLACEMENT_3D ( 'NONE', #126336, #105405, #106681 ) ;
#125459=ADVANCED_FACE ( 'NONE', ( #70688 ), #60867, .T. ) ;
#125460=DIRECTION ( 'NONE',  ( 0.000000000000000000, 0.000000000000000000, 1.000000000000000000 ) ) ;
#125461=CONICAL_SURFACE ( 'NONE', #110790, 0.09999999999999982514, 0.003490658503988666988 ) ;
#125462=DIRECTION ( 'NONE',  ( -0.000000000000000000, 1.000000000000000000, -0.000000000000000000 ) ) ;
#125463=DIRECTION ( 'NONE',  ( 0.000000000000000000, 0.000000000000000000, 1.000000000000000000 ) ) ;
#125464=ORIENTED_EDGE ( 'NONE', *, *, #14129, .F. ) ;
#125465=VERTEX_POINT ( 'NONE', #90308 ) ;
#125466=FACE_OUTER_BOUND ( 'NONE', #89844, .T. ) ;
#125467=AXIS2_PLACEMENT_3D ( 'NONE', #110574, #20262, #60210 ) ;
#125468=VERTEX_POINT ( 'NONE', #649 ) ;
#125469=DIRECTION ( 'NONE',  ( 0.000000000000000000, 0.000000000000000000, 1.000000000000000000 ) ) ;
#125470=FACE_OUTER_BOUND ( 'NONE', #18219, .T. ) ;
#125471=EDGE_LOOP ( 'NONE', ( #52908, #57803, #92770, #56181 ) ) ;
#125472=DIRECTION ( 'NONE',  ( -4.274815082592931898E-19, -0.9999939076577903929, -0.003490651415223739937 ) ) ;
#125473=DIRECTION ( 'NONE',  ( -4.274815082592931898E-19, -0.9999939076577903929, -0.003490651415223739937 ) ) ;
#125474=CONICAL_SURFACE ( 'NONE', #81, 0.1000000000000000472, 0.003490658503988666988 ) ;
#125475=DIRECTION ( 'NONE',  ( 0.000000000000000000, 0.000000000000000000, 1.000000000000000000 ) ) ;
#125476=EDGE_CURVE ( 'NONE', #35640, #71388, #6774, .T. ) ;
#125477=EDGE_CURVE ( 'NONE', #9409, #85421, #8843, .T. ) ;
#125478=DIRECTION ( 'NONE',  ( -0.000000000000000000, -1.000000000000000000, -0.000000000000000000 ) ) ;
#125479=VERTEX_POINT ( 'NONE', #92923 ) ;
#125480=PLANE ( 'NONE',  #96838 ) ;
#125482=ORIENTED_EDGE ( 'NONE', *, *, #4632, .F. ) ;
#125484=EDGE_LOOP ( 'NONE', ( #65161, #23710, #111729, #35900 ) ) ;
#125485=EDGE_CURVE ( 'NONE', #7764, #111299, #112559, .T. ) ;
#125487=DIRECTION ( 'NONE',  ( 0.000000000000000000, 0.000000000000000000, 1.000000000000000000 ) ) ;
#125488=DIRECTION ( 'NONE',  ( -0.000000000000000000, 1.000000000000000000, -0.000000000000000000 ) ) ;
#125489=CARTESIAN_POINT ( 'NONE',  ( 14.99999999999989342, 12.50000000000000000, -0.6277270498435166823 ) ) ;
#125490=CARTESIAN_POINT ( 'NONE',  ( -12.49999999999999467, 2.500000000000000000, 0.7928203230275536750 ) ) ;
#125491=CARTESIAN_POINT ( 'NONE',  ( 10.39999999999991154, 2.500000000000000000, -5.022947341949754119 ) ) ;
#125493=PLANE ( 'NONE',  #95047 ) ;
#125494=DIRECTION ( 'NONE',  ( 0.000000000000000000, 0.000000000000000000, 1.000000000000000000 ) ) ;
#125495=CIRCLE ( 'NONE', #110822, 0.06509327318403745899 ) ;
#125496=CONICAL_SURFACE ( 'NONE', #56535, 0.1000000000000000472, 0.003490658503988666988 ) ;
#125497=FACE_OUTER_BOUND ( 'NONE', #32956, .T. ) ;
#125498=VERTEX_POINT ( 'NONE', #81781 ) ;
#125499=AXIS2_PLACEMENT_3D ( 'NONE', #69655, #108920, #111512 ) ;
#125500=CIRCLE ( 'NONE', #41897, 0.1000000000000002554 ) ;
#125501=ORIENTED_EDGE ( 'NONE', *, *, #36045, .T. ) ;
#125502=VERTEX_POINT ( 'NONE', #101443 ) ;
#125503=CARTESIAN_POINT ( 'NONE',  ( 8.149999999999923972, 2.500000000000000000, -6.841600689897077814 ) ) ;
#125504=DIRECTION ( 'NONE',  ( 0.000000000000000000, -0.9999939076577903929, 0.003490651415223739937 ) ) ;
#125506=EDGE_LOOP ( 'NONE', ( #80555, #97938, #84940, #41457 ) ) ;
#125507=CARTESIAN_POINT ( 'NONE',  ( -5.850000000000019185, 2.500000000000000000, 6.595190528383296780 ) ) ;
#125508=ADVANCED_FACE ( 'NONE', ( #51068 ), #54820, .T. ) ;
#125510=LINE ( 'NONE', #35853, #129612 ) ;
#125511=ORIENTED_EDGE ( 'NONE', *, *, #68865, .F. ) ;
#125512=EDGE_CURVE ( 'NONE', #69417, #63398, #21376, .T. ) ;
#125513=EDGE_CURVE ( 'NONE', #119556, #18789, #125921, .T. ) ;
#125514=CARTESIAN_POINT ( 'NONE',  ( 9.199999999999915801, 2.500000000000000000, 4.330127018922196314 ) ) ;
#125515=ORIENTED_EDGE ( 'NONE', *, *, #41680, .T. ) ;
#125516=ORIENTED_EDGE ( 'NONE', *, *, #20970, .F. ) ;
#125517=EDGE_LOOP ( 'NONE', ( #48335, #111396 ) ) ;
#125518=ORIENTED_EDGE ( 'NONE', *, *, #85313, .F. ) ;
#125519=CARTESIAN_POINT ( 'NONE',  ( -9.550000000000002487, 2.500000000000000000, 6.395190528383296602 ) ) ;
#125520=EDGE_CURVE ( 'NONE', #77155, #101605, #100779, .T. ) ;
#125521=EDGE_CURVE ( 'NONE', #31027, #64400, #63239, .T. ) ;
#125522=EDGE_CURVE ( 'NONE', #19669, #7901, #22894, .T. ) ;
#125523=CARTESIAN_POINT ( 'NONE',  ( 9.349999999999916156, 12.50000000000000000, -2.511473670974877948 ) ) ;
#125524=CARTESIAN_POINT ( 'NONE',  ( -11.84999999999999787, 2.500000000000000000, -6.148780366869522673 ) ) ;
#125525=CARTESIAN_POINT ( 'NONE',  ( -4.150000000000025224, 2.500000000000000000, -1.572243186433550211 ) ) ;
#125526=AXIS2_PLACEMENT_3D ( 'NONE', #79315, #69462, #59686 ) ;
#125527=VERTEX_POINT ( 'NONE', #92249 ) ;
#125528=EDGE_CURVE ( 'NONE', #79994, #30131, #77804, .T. ) ;
#125529=DIRECTION ( 'NONE',  ( 0.000000000000000000, 1.000000000000000000, 0.000000000000000000 ) ) ;
#125530=VERTEX_POINT ( 'NONE', #41890 ) ;
#125531=CARTESIAN_POINT ( 'NONE',  ( -4.077611073288324453E-14, 12.50000000000000000, -5.088040615133791356 ) ) ;
#125532=DIRECTION ( 'NONE',  ( 0.000000000000000000, 0.000000000000000000, -1.000000000000000000 ) ) ;
#125533=DIRECTION ( 'NONE',  ( -0.000000000000000000, -1.000000000000000000, -0.000000000000000000 ) ) ;
#125534=CARTESIAN_POINT ( 'NONE',  ( 18.20334136263782199, -2.532871263996936406, 4.817802756298863898 ) ) ;
#125535=AXIS2_PLACEMENT_3D ( 'NONE', #54682, #3040, #103163 ) ;
#125536=ADVANCED_FACE ( 'NONE', ( #82462 ), #96667, .T. ) ;
#125537=EDGE_LOOP ( 'NONE', ( #55075, #126118, #7292, #17407 ) ) ;
#125538=VERTEX_POINT ( 'NONE', #102707 ) ;
#125539=EDGE_LOOP ( 'NONE', ( #47317, #117254, #125087, #85792 ) ) ;
#125540=CARTESIAN_POINT ( 'NONE',  ( -2.300000000000033573, 2.500000000000000000, -3.883716857408426648 ) ) ;
#125541=DIRECTION ( 'NONE',  ( 0.000000000000000000, -0.000000000000000000, 1.000000000000000000 ) ) ;
#125542=FACE_OUTER_BOUND ( 'NONE', #55241, .T. ) ;
#125543=FACE_BOUND ( 'NONE', #27472, .T. ) ;
#125544=DIRECTION ( 'NONE',  ( 0.000000000000000000, -0.9999939076577903929, 0.003490651415223739937 ) ) ;
#125545=CARTESIAN_POINT ( 'NONE',  ( -7.500000000000001776, -1.500000000000000000, 1.734723475976807094E-15 ) ) ;
#125546=CARTESIAN_POINT ( 'NONE',  ( -5.650000000000019895, 12.50000000000000000, 1.818653347947321475 ) ) ;
#125548=CONICAL_SURFACE ( 'NONE', #52396, 0.1000000000000000056, 0.003490658503988666988 ) ;
#125550=DIRECTION ( 'NONE',  ( -4.274815082592931898E-19, -0.9999939076577903929, -0.003490651415223739937 ) ) ;
#125551=CARTESIAN_POINT ( 'NONE',  ( 11.44999999999990514, 12.50000000000000000, 2.576566944158910744 ) ) ;
#125552=AXIS2_PLACEMENT_3D ( 'NONE', #14915, #75167, #67234 ) ;
#125553=FACE_OUTER_BOUND ( 'NONE', #18102, .T. ) ;
#125554=ORIENTED_EDGE ( 'NONE', *, *, #21382, .F. ) ;
#125555=CIRCLE ( 'NONE', #35694, 0.09999999999999982514 ) ;
#125556=ORIENTED_EDGE ( 'NONE', *, *, #24324, .T. ) ;
#125557=EDGE_LOOP ( 'NONE', ( #91959, #54112, #46242, #62986 ) ) ;
#125558=ORIENTED_EDGE ( 'NONE', *, *, #55045, .T. ) ;
#125559=DIRECTION ( 'NONE',  ( 0.000000000000000000, 0.000000000000000000, 1.000000000000000000 ) ) ;
#125560=FACE_BOUND ( 'NONE', #15097, .T. ) ;
#125561=CARTESIAN_POINT ( 'NONE',  ( 1.699999999999951994, 2.500000000000000000, -4.430127018922202176 ) ) ;
#125562=ADVANCED_FACE ( 'NONE', ( #43184 ), #83100, .T. ) ;
#125563=EDGE_LOOP ( 'NONE', ( #58605, #16598 ) ) ;
#125564=DIRECTION ( 'NONE',  ( -0.000000000000000000, -1.000000000000000000, -0.000000000000000000 ) ) ;
#125565=DIRECTION ( 'NONE',  ( 0.000000000000000000, 0.000000000000000000, 1.000000000000000000 ) ) ;
#125566=ORIENTED_EDGE ( 'NONE', *, *, #85848, .F. ) ;
#125567=CARTESIAN_POINT ( 'NONE',  ( -14.14999999999998614, 2.500000000000000000, -2.757883832488651876 ) ) ;
#125568=FACE_OUTER_BOUND ( 'NONE', #75049, .T. ) ;
#125569=EDGE_CURVE ( 'NONE', #108133, #126539, #23520, .T. ) ;
#125570=AXIS2_PLACEMENT_3D ( 'NONE', #43241, #43883, #123073 ) ;
#125571=ORIENTED_EDGE ( 'NONE', *, *, #121700, .T. ) ;
#125572=CONICAL_SURFACE ( 'NONE', #54484, 0.09999999999999982514, 0.003490658503988666988 ) ;
#125573=CARTESIAN_POINT ( 'NONE',  ( -11.25000000000000000, 2.500000000000000000, 2.857883832488649301 ) ) ;
#125574=CIRCLE ( 'NONE', #44112, 0.1000000000000000056 ) ;
#125575=CARTESIAN_POINT ( 'NONE',  ( -5.450000000000019718, 12.50000000000000000, 6.560283801567334372 ) ) ;
#125576=EDGE_LOOP ( 'NONE', ( #26488, #78472 ) ) ;
#125577=DIRECTION ( 'NONE',  ( 0.000000000000000000, 0.000000000000000000, -1.000000000000000000 ) ) ;
#125578=VECTOR ( 'NONE', #68207, 1000.000000000000000 ) ;
#125579=DIRECTION ( 'NONE',  ( -0.000000000000000000, -1.000000000000000000, -0.000000000000000000 ) ) ;
#125580=ORIENTED_EDGE ( 'NONE', *, *, #15560, .T. ) ;
#125581=DIRECTION ( 'NONE',  ( 0.000000000000000000, 1.000000000000000000, 0.000000000000000000 ) ) ;
#125582=EDGE_LOOP ( 'NONE', ( #95200, #79495 ) ) ;
#125583=CIRCLE ( 'NONE', #90076, 0.06509327318403745899 ) ;
#125584=ORIENTED_EDGE ( 'NONE', *, *, #38304, .T. ) ;
#125586=VERTEX_POINT ( 'NONE', #104020 ) ;
#125587=LINE ( 'NONE', #94210, #86708 ) ;
#125588=DIRECTION ( 'NONE',  ( -0.000000000000000000, -1.000000000000000000, -0.000000000000000000 ) ) ;
#125589=ORIENTED_EDGE ( 'NONE', *, *, #23639, .F. ) ;
#125590=CARTESIAN_POINT ( 'NONE',  ( 1.649999999999949729, 12.50000000000000000, 5.802370205355744659 ) ) ;
#125591=DIRECTION ( 'NONE',  ( 0.000000000000000000, -0.9999939076577903929, 0.003490651415223739937 ) ) ;
#125592=DIRECTION ( 'NONE',  ( -0.000000000000000000, -1.000000000000000000, -0.000000000000000000 ) ) ;
#125593=DIRECTION ( 'NONE',  ( 0.000000000000000000, 0.000000000000000000, 1.000000000000000000 ) ) ;
#125594=DIRECTION ( 'NONE',  ( 0.000000000000000000, 0.000000000000000000, 1.000000000000000000 ) ) ;
#125595=CARTESIAN_POINT ( 'NONE',  ( 17.48308156489505549, 2.102418598454959486, -4.293689242909686676 ) ) ;
#125596=VERTEX_POINT ( 'NONE', #26108 ) ;
#125597=EDGE_CURVE ( 'NONE', #97446, #11600, #533, .T. ) ;
#125598=VERTEX_POINT ( 'NONE', #113179 ) ;
#125599=AXIS2_PLACEMENT_3D ( 'NONE', #23532, #44467, #55583 ) ;
#125600=FACE_OUTER_BOUND ( 'NONE', #46884, .T. ) ;
#125601=CARTESIAN_POINT ( 'NONE',  ( -1.050000000000037792, 2.500000000000000000, 1.818653347947321475 ) ) ;
#125602=CARTESIAN_POINT ( 'NONE',  ( -14.34999999999998543, 2.500000000000000000, 2.511473670974877503 ) ) ;
#125603=ORIENTED_EDGE ( 'NONE', *, *, #75871, .F. ) ;
#125604=ORIENTED_EDGE ( 'NONE', *, *, #41554, .F. ) ;
#125605=EDGE_LOOP ( 'NONE', ( #21444, #115281, #53811, #62690 ) ) ;
#125606=ADVANCED_FACE ( 'NONE', ( #105948 ), #45108, .T. ) ;
#125607=LINE ( 'NONE', #16918, #114885 ) ;
#125608=AXIS2_PLACEMENT_3D ( 'NONE', #121636, #92174, #109902 ) ;
#125609=DIRECTION ( 'NONE',  ( -0.000000000000000000, -1.000000000000000000, -0.000000000000000000 ) ) ;
#125610=ADVANCED_FACE ( 'NONE', ( #104644 ), #27621, .T. ) ;
#125611=DIRECTION ( 'NONE',  ( 0.000000000000000000, 1.000000000000000000, 0.000000000000000000 ) ) ;
#125613=FACE_OUTER_BOUND ( 'NONE', #75371, .T. ) ;
#125614=CARTESIAN_POINT ( 'NONE',  ( -10.40000000000000391, 12.50000000000000000, -3.572213422710607933 ) ) ;
#125615=FACE_OUTER_BOUND ( 'NONE', #71780, .T. ) ;
#125616=DIRECTION ( 'NONE',  ( 0.000000000000000000, 0.000000000000000000, 1.000000000000000000 ) ) ;
#125617=LINE ( 'NONE', #117724, #46717 ) ;
#125618=ADVANCED_FACE ( 'NONE', ( #44451 ), #56957, .T. ) ;
#125619=ADVANCED_FACE ( 'NONE', ( #86290 ), #53629, .T. ) ;
#125620=CARTESIAN_POINT ( 'NONE',  ( 6.449999999999930012, 2.500000000000000000, 1.918653347947321564 ) ) ;
#125621=CONICAL_SURFACE ( 'NONE', #19004, 0.09999999999999982514, 0.003490658503988666988 ) ;
#125622=CONICAL_SURFACE ( 'NONE', #21072, 0.1000000000000002554, 0.003490658503988666988 ) ;
#125623=ORIENTED_EDGE ( 'NONE', *, *, #29583, .F. ) ;
#125624=ADVANCED_FACE ( 'NONE', ( #65367 ), #48581, .T. ) ;
#125625=DIRECTION ( 'NONE',  ( 0.000000000000000000, 0.000000000000000000, 1.000000000000000000 ) ) ;
#125626=VERTEX_POINT ( 'NONE', #93552 ) ;
#125627=EDGE_LOOP ( 'NONE', ( #107488, #123149 ) ) ;
#125628=EDGE_CURVE ( 'NONE', #85037, #102865, #59045, .T. ) ;
#125629=CARTESIAN_POINT ( 'NONE',  ( 6.899999999999926636, 2.500000000000000000, 0.3464101615137736845 ) ) ;
#125630=FACE_OUTER_BOUND ( 'NONE', #71303, .T. ) ;
#125631=CARTESIAN_POINT ( 'NONE',  ( -6.250000000000021316, 2.500000000000000000, -1.472243186433550122 ) ) ;
#125632=CONICAL_SURFACE ( 'NONE', #113027, 0.1000000000000002554, 0.003490658503988666988 ) ;
#125633=DIRECTION ( 'NONE',  ( 0.000000000000000000, -0.9999939076577903929, 0.003490651415223739937 ) ) ;
#125634=CIRCLE ( 'NONE', #39898, 0.09999999999999982514 ) ;
#125635=DIRECTION ( 'NONE',  ( -0.000000000000000000, -1.000000000000000000, -0.000000000000000000 ) ) ;
#125636=DIRECTION ( 'NONE',  ( 0.000000000000000000, 1.000000000000000000, 0.000000000000000000 ) ) ;
#125637=CARTESIAN_POINT ( 'NONE',  ( 11.84999999999990727, 2.500000000000000000, -1.918653347947326004 ) ) ;
#125638=ORIENTED_EDGE ( 'NONE', *, *, #22311, .T. ) ;
#125639=CARTESIAN_POINT ( 'NONE',  ( 10.44999999999991047, 2.500000000000000000, 2.165063509461097713 ) ) ;
#125640=AXIS2_PLACEMENT_3D ( 'NONE', #123450, #93361, #42329 ) ;
#125641=PLANE ( 'NONE',  #87494 ) ;
#125642=EDGE_LOOP ( 'NONE', ( #32604, #110432, #18, #95057 ) ) ;
#125643=EDGE_LOOP ( 'NONE', ( #15552, #9270, #89974, #32865 ) ) ;
#125644=AXIS2_PLACEMENT_3D ( 'NONE', #38411, #97311, #78333 ) ;
#125645=VERTEX_POINT ( 'NONE', #84376 ) ;
#125646=ORIENTED_EDGE ( 'NONE', *, *, #94919, .T. ) ;
#125647=DIRECTION ( 'NONE',  ( 0.000000000000000000, 1.000000000000000000, 0.000000000000000000 ) ) ;
#125648=DIRECTION ( 'NONE',  ( 0.000000000000000000, 0.000000000000000000, -1.000000000000000000 ) ) ;
#125649=PLANE ( 'NONE',  #12979 ) ;
#125650=CARTESIAN_POINT ( 'NONE',  ( 0.8499999999999553468, 2.500000000000000000, 2.065063509461097624 ) ) ;
#125651=DIRECTION ( 'NONE',  ( -4.274815082592931898E-19, -0.9999939076577903929, -0.003490651415223739937 ) ) ;
#125652=ORIENTED_EDGE ( 'NONE', *, *, #50639, .T. ) ;
#125653=DIRECTION ( 'NONE',  ( 0.000000000000000000, 1.000000000000000000, 0.000000000000000000 ) ) ;
#125654=ADVANCED_FACE ( 'NONE', ( #14951 ), #124303, .T. ) ;
#125655=DIRECTION ( 'NONE',  ( 0.000000000000000000, -0.9999939076577903929, 0.003490651415223739937 ) ) ;
#125656=EDGE_LOOP ( 'NONE', ( #89548, #11354, #102663, #38504 ) ) ;
#125657=VERTEX_POINT ( 'NONE', #74554 ) ;
#125658=EDGE_LOOP ( 'NONE', ( #45519, #119858, #51505, #126976 ) ) ;
#125659=AXIS2_PLACEMENT_3D ( 'NONE', #96172, #94897, #77192 ) ;
#125660=EDGE_CURVE ( 'NONE', #43024, #88967, #73689, .T. ) ;
#125661=DIRECTION ( 'NONE',  ( 0.000000000000000000, 0.000000000000000000, 1.000000000000000000 ) ) ;
#125662=AXIS2_PLACEMENT_3D ( 'NONE', #110676, #70129, #50473 ) ;
#125663=ADVANCED_FACE ( 'NONE', ( #96122 ), #42317, .T. ) ;
#125664=ADVANCED_FACE ( 'NONE', ( #94842 ), #33998, .T. ) ;
#125665=EDGE_CURVE ( 'NONE', #13889, #127971, #2576, .T. ) ;
#125667=CARTESIAN_POINT ( 'NONE',  ( -10.85000000000000142, 2.500000000000000000, -6.595190528383298556 ) ) ;
#125668=CIRCLE ( 'NONE', #69235, 0.1000000000000002554 ) ;
#125669=CIRCLE ( 'NONE', #12796, 0.09999999999999982514 ) ;
#125670=EDGE_CURVE ( 'NONE', #74953, #19040, #83735, .T. ) ;
#125671=ORIENTED_EDGE ( 'NONE', *, *, #97604, .F. ) ;
#125672=DIRECTION ( 'NONE',  ( 0.000000000000000000, 0.000000000000000000, 1.000000000000000000 ) ) ;
#125673=FACE_OUTER_BOUND ( 'NONE', #19370, .T. ) ;
#125674=CARTESIAN_POINT ( 'NONE',  ( -6.250000000000019540, 2.500000000000000000, -2.857883832488653741 ) ) ;
#125676=CARTESIAN_POINT ( 'NONE',  ( 8.149999999999920419, 2.500000000000000000, -1.818653347947325916 ) ) ;
#125677=EDGE_CURVE ( 'NONE', #101819, #110619, #109198, .T. ) ;
#125678=VERTEX_POINT ( 'NONE', #103377 ) ;
#125679=ADVANCED_FACE ( 'NONE', ( #16880 ), #77759, .T. ) ;
#125680=DIRECTION ( 'NONE',  ( 0.000000000000000000, 0.000000000000000000, -1.000000000000000000 ) ) ;
#125681=VERTEX_POINT ( 'NONE', #8381 ) ;
#125682=VERTEX_POINT ( 'NONE', #29337 ) ;
#125683=EDGE_LOOP ( 'NONE', ( #30821, #55489, #33397, #120945 ) ) ;
#125684=CARTESIAN_POINT ( 'NONE',  ( -9.800000000000006040, 2.500000000000000000, 4.676537180435972552 ) ) ;
#125685=FACE_BOUND ( 'NONE', #92714, .T. ) ;
#125686=CARTESIAN_POINT ( 'NONE',  ( -3.350000000000028511, 12.50000000000000000, -2.922977105672691422 ) ) ;
#125687=DIRECTION ( 'NONE',  ( -0.000000000000000000, 1.000000000000000000, -0.000000000000000000 ) ) ;
#125688=DIRECTION ( 'NONE',  ( 0.000000000000000000, 0.000000000000000000, -1.000000000000000000 ) ) ;
#125689=ORIENTED_EDGE ( 'NONE', *, *, #14711, .T. ) ;
#125690=DIRECTION ( 'NONE',  ( -0.000000000000000000, 1.000000000000000000, -0.000000000000000000 ) ) ;
#125691=DIRECTION ( 'NONE',  ( 0.000000000000000000, -0.9999939076577903929, 0.003490651415223739937 ) ) ;
#125692=CARTESIAN_POINT ( 'NONE',  ( -7.900000000000011013, 12.50000000000000000, 3.637306695894644726 ) ) ;
#125693=DIRECTION ( 'NONE',  ( 0.000000000000000000, 1.000000000000000000, 0.000000000000000000 ) ) ;
#125694=ORIENTED_EDGE ( 'NONE', *, *, #52619, .F. ) ;
#125695=CONICAL_SURFACE ( 'NONE', #29570, 0.09999999999999982514, 0.003490658503988666988 ) ;
#125696=CARTESIAN_POINT ( 'NONE',  ( 1.849999999999949019, 12.50000000000000000, 6.776507416713035248 ) ) ;
#125697=DIRECTION ( 'NONE',  ( -0.000000000000000000, -1.000000000000000000, -0.000000000000000000 ) ) ;
#125698=EDGE_LOOP ( 'NONE', ( #67776, #59796 ) ) ;
#125699=DIRECTION ( 'NONE',  ( 0.000000000000000000, -0.000000000000000000, 1.000000000000000000 ) ) ;
#125700=FACE_BOUND ( 'NONE', #99058, .T. ) ;
#125701=CIRCLE ( 'NONE', #54687, 0.06509327318403745899 ) ;
#125703=AXIS2_PLACEMENT_3D ( 'NONE', #88952, #78507, #28751 ) ;
#125704=VERTEX_POINT ( 'NONE', #99363 ) ;
#125705=PLANE ( 'NONE',  #65361 ) ;
#125706=DIRECTION ( 'NONE',  ( -0.000000000000000000, 1.000000000000000000, -0.000000000000000000 ) ) ;
#125707=EDGE_LOOP ( 'NONE', ( #71985, #41816, #107440, #91039 ) ) ;
#125708=VERTEX_POINT ( 'NONE', #107234 ) ;
#125711=EDGE_LOOP ( 'NONE', ( #58321, #32106 ) ) ;
#125714=DIRECTION ( 'NONE',  ( 0.000000000000000000, -0.000000000000000000, 1.000000000000000000 ) ) ;
#125715=ADVANCED_FACE ( 'NONE', ( #118343 ), #7083, .T. ) ;
#125716=DIRECTION ( 'NONE',  ( 0.000000000000000000, 0.000000000000000000, -1.000000000000000000 ) ) ;
#125717=CIRCLE ( 'NONE', #65083, 0.09999999999999982514 ) ;
#125718=LINE ( 'NONE', #104168, #75994 ) ;
#125719=CARTESIAN_POINT ( 'NONE',  ( -6.650000000000018119, 12.50000000000000000, -2.165063509461101710 ) ) ;
#125720=AXIS2_PLACEMENT_3D ( 'NONE', #92552, #72920, #23164 ) ;
#125721=ORIENTED_EDGE ( 'NONE', *, *, #98551, .F. ) ;
#125722=ORIENTED_EDGE ( 'NONE', *, *, #120009, .F. ) ;
#125723=CARTESIAN_POINT ( 'NONE',  ( 1.249999999999988898, 12.50000000000000000, -6.495190528383302464 ) ) ;
#125724=AXIS2_PLACEMENT_3D ( 'NONE', #127203, #60404, #98355 ) ;
#125725=AXIS2_PLACEMENT_3D ( 'NONE', #80899, #40335, #90050 ) ;
#125726=CARTESIAN_POINT ( 'NONE',  ( -4.150000000000024336, 2.500000000000000000, 2.265063509461097357 ) ) ;
#125727=CARTESIAN_POINT ( 'NONE',  ( -8.150000000000012790, 12.50000000000000000, 2.511473670974873507 ) ) ;
#125728=DIRECTION ( 'NONE',  ( 0.000000000000000000, 0.000000000000000000, -1.000000000000000000 ) ) ;
#125729=EDGE_LOOP ( 'NONE', ( #46674, #47022 ) ) ;
#125730=ORIENTED_EDGE ( 'NONE', *, *, #86939, .T. ) ;
#125731=CARTESIAN_POINT ( 'NONE',  ( -8.550000000000014921, 2.500000000000000000, -6.148780366869520897 ) ) ;
#125732=VERTEX_POINT ( 'NONE', #117674 ) ;
#125733=DIRECTION ( 'NONE',  ( 0.000000000000000000, -0.000000000000000000, 1.000000000000000000 ) ) ;
#125734=DIRECTION ( 'NONE',  ( 0.000000000000000000, 1.000000000000000000, 0.000000000000000000 ) ) ;
#125735=EDGE_LOOP ( 'NONE', ( #50962, #34500, #118419, #50923 ) ) ;
#125736=CARTESIAN_POINT ( 'NONE',  ( 5.199999999999937117, 12.50000000000000000, -4.676537180435978769 ) ) ;
#125737=LINE ( 'NONE', #7253, #62007 ) ;
#125738=DIRECTION ( 'NONE',  ( -0.000000000000000000, 1.000000000000000000, -0.000000000000000000 ) ) ;
#125739=DIRECTION ( 'NONE',  ( 0.000000000000000000, 1.000000000000000000, 0.000000000000000000 ) ) ;
#125740=DIRECTION ( 'NONE',  ( 0.000000000000000000, 0.000000000000000000, -1.000000000000000000 ) ) ;
#125741=DIRECTION ( 'NONE',  ( -0.000000000000000000, -1.000000000000000000, -0.000000000000000000 ) ) ;
#125742=CARTESIAN_POINT ( 'NONE',  ( -5.600000000000020073, 2.500000000000000000, 4.676537180435972552 ) ) ;
#125743=DIRECTION ( 'NONE',  ( -0.000000000000000000, 1.000000000000000000, -0.000000000000000000 ) ) ;
#125744=DIRECTION ( 'NONE',  ( -0.000000000000000000, 1.000000000000000000, -0.000000000000000000 ) ) ;
#125745=ORIENTED_EDGE ( 'NONE', *, *, #54879, .T. ) ;
#125746=ORIENTED_EDGE ( 'NONE', *, *, #94665, .F. ) ;
#125747=DIRECTION ( 'NONE',  ( -0.000000000000000000, 1.000000000000000000, -0.000000000000000000 ) ) ;
#125748=ORIENTED_EDGE ( 'NONE', *, *, #52839, .F. ) ;
#125749=AXIS2_PLACEMENT_3D ( 'NONE', #127643, #97531, #7858 ) ;
#125750=DIRECTION ( 'NONE',  ( 0.000000000000000000, 0.000000000000000000, 1.000000000000000000 ) ) ;
#125751=AXIS2_PLACEMENT_3D ( 'NONE', #65278, #105211, #35833 ) ;
#125752=VERTEX_POINT ( 'NONE', #49627 ) ;
#125753=ORIENTED_EDGE ( 'NONE', *, *, #18173, .T. ) ;
#125754=ORIENTED_EDGE ( 'NONE', *, *, #56730, .T. ) ;
#125755=DIRECTION ( 'NONE',  ( 0.000000000000000000, -0.000000000000000000, 1.000000000000000000 ) ) ;
#125756=ADVANCED_FACE ( 'NONE', ( #128178 ), #88350, .T. ) ;
#125757=AXIS2_PLACEMENT_3D ( 'NONE', #123597, #111865, #102670 ) ;
#125758=CARTESIAN_POINT ( 'NONE',  ( -5.850000000000022737, 12.50000000000000000, -6.560283801567339701 ) ) ;
#125759=CIRCLE ( 'NONE', #96509, 0.09999999999999999167 ) ;
#125760=DIRECTION ( 'NONE',  ( 0.000000000000000000, 0.000000000000000000, 1.000000000000000000 ) ) ;
#125761=FACE_OUTER_BOUND ( 'NONE', #30123, .T. ) ;
#125762=CIRCLE ( 'NONE', #27564, 0.06509327318403745899 ) ;
#125763=CARTESIAN_POINT ( 'NONE',  ( -0.8500000000000386136, 12.50000000000000000, 7.122917578226811486 ) ) ;
#125764=AXIS2_PLACEMENT_3D ( 'NONE', #63068, #94447, #4767 ) ;
#125765=EDGE_CURVE ( 'NONE', #124238, #98747, #57501, .T. ) ;
#125766=ORIENTED_EDGE ( 'NONE', *, *, #9047, .F. ) ;
#125767=EDGE_CURVE ( 'NONE', #45092, #15933, #76498, .T. ) ;
#125768=DIRECTION ( 'NONE',  ( -4.274815082592931898E-19, -0.9999939076577903929, -0.003490651415223739937 ) ) ;
#125769=CIRCLE ( 'NONE', #79816, 0.06509327318403745899 ) ;
#125770=EDGE_LOOP ( 'NONE', ( #110284, #56015 ) ) ;
#125771=EDGE_LOOP ( 'NONE', ( #101788, #82119 ) ) ;
#125772=ORIENTED_EDGE ( 'NONE', *, *, #65859, .T. ) ;
#125773=ORIENTED_EDGE ( 'NONE', *, *, #42138, .F. ) ;
#125774=ADVANCED_FACE ( 'NONE', ( #116398 ), #42421, .T. ) ;
#125775=CARTESIAN_POINT ( 'NONE',  ( 3.099999999999943245, 2.500000000000000000, 3.983716857408420076 ) ) ;
#125776=EDGE_CURVE ( 'NONE', #56169, #88605, #61187, .T. ) ;
#125777=EDGE_CURVE ( 'NONE', #7618, #43527, #54911, .T. ) ;
#125778=ORIENTED_EDGE ( 'NONE', *, *, #95048, .F. ) ;
#125779=EDGE_LOOP ( 'NONE', ( #9333, #122204 ) ) ;
#125780=ADVANCED_FACE ( 'NONE', ( #69230 ), #19402, .T. ) ;
#125781=DIRECTION ( 'NONE',  ( 0.000000000000000000, 0.000000000000000000, -1.000000000000000000 ) ) ;
#125782=CARTESIAN_POINT ( 'NONE',  ( 10.39999999999990976, 2.500000000000000000, 4.330127018922196314 ) ) ;
#125783=PLANE ( 'NONE',  #67244 ) ;
#125784=PLANE ( 'NONE',  #17832 ) ;
#125785=B_SPLINE_CURVE_WITH_KNOTS ( 'NONE', 3,
 ( #85686, #35951, #127554, #85040, #117066, #75225, #37882, #65398, #26775, #86322, #37255, #16913 ),
 .UNSPECIFIED., .F., .F.,
 ( 4, 2, 2, 2, 2, 4 ),
 ( 8.673617379884035472E-19, 0.0006571239767409088736, 0.001314247953481816880, 0.002628495906963632892, 0.003942743860445448688, 0.005256991813927264917 ),
 .UNSPECIFIED. ) ;
#125786=CARTESIAN_POINT ( 'NONE',  ( -7.100000000000018296, 12.50000000000000000, -2.385244779468109755E-15 ) ) ;
#125787=ORIENTED_EDGE ( 'NONE', *, *, #2313, .F. ) ;
#125788=ADVANCED_FACE ( 'NONE', ( #37223 ), #59145, .T. ) ;
#125789=DIRECTION ( 'NONE',  ( 0.000000000000000000, 0.000000000000000000, -1.000000000000000000 ) ) ;
#125790=AXIS2_PLACEMENT_3D ( 'NONE', #109744, #80932, #120845 ) ;
#125791=AXIS2_PLACEMENT_3D ( 'NONE', #99587, #119857, #29547 ) ;
#125792=VERTEX_POINT ( 'NONE', #88888 ) ;
#125793=DIRECTION ( 'NONE',  ( -0.000000000000000000, -1.000000000000000000, -0.000000000000000000 ) ) ;
#125794=ORIENTED_EDGE ( 'NONE', *, *, #122856, .F. ) ;
#125795=DIRECTION ( 'NONE',  ( -0.000000000000000000, -1.000000000000000000, -0.000000000000000000 ) ) ;
#125796=ORIENTED_EDGE ( 'NONE', *, *, #20049, .F. ) ;
#125797=ORIENTED_EDGE ( 'NONE', *, *, #42034, .T. ) ;
#125798=AXIS2_PLACEMENT_3D ( 'NONE', #48929, #88834, #128792 ) ;
#125799=DIRECTION ( 'NONE',  ( 0.000000000000000000, -0.000000000000000000, 1.000000000000000000 ) ) ;
#125800=CARTESIAN_POINT ( 'NONE',  ( -8.350000000000008527, 2.500000000000000000, 7.188010851410848723 ) ) ;
#125801=CIRCLE ( 'NONE', #38088, 0.06509327318403745899 ) ;
#125802=CIRCLE ( 'NONE', #2468, 0.06509327318403745899 ) ;
#125804=CIRCLE ( 'NONE', #86082, 0.1000000000000002554 ) ;
#125806=CARTESIAN_POINT ( 'NONE',  ( 7.099999999999927702, 2.500000000000000000, -3.637306695894650055 ) ) ;
#125807=CARTESIAN_POINT ( 'NONE',  ( -5.650000000000023448, 12.50000000000000000, -2.576566944158915184 ) ) ;
#125808=ORIENTED_EDGE ( 'NONE', *, *, #22511, .F. ) ;
#125809=DIRECTION ( 'NONE',  ( 0.000000000000000000, 1.000000000000000000, 0.000000000000000000 ) ) ;
#125810=CARTESIAN_POINT ( 'NONE',  ( -11.24999999999999822, 2.500000000000000000, 5.702370205355745014 ) ) ;
#125811=ADVANCED_FACE ( 'NONE', ( #18201 ), #71647, .T. ) ;
#125812=DIRECTION ( 'NONE',  ( 0.000000000000000000, 0.000000000000000000, -1.000000000000000000 ) ) ;
#125813=CARTESIAN_POINT ( 'NONE',  ( 11.64999999999990798, 12.50000000000000000, 5.867463478539781896 ) ) ;
#125815=AXIS2_PLACEMENT_3D ( 'NONE', #15913, #2892, #122659 ) ;
#125816=DIRECTION ( 'NONE',  ( -0.000000000000000000, -1.000000000000000000, -0.000000000000000000 ) ) ;
#125817=ORIENTED_EDGE ( 'NONE', *, *, #124857, .T. ) ;
#125818=AXIS2_PLACEMENT_3D ( 'NONE', #92560, #2900, #42852 ) ;
#125819=CONICAL_SURFACE ( 'NONE', #33899, 0.1000000000000002554, 0.003490658503988666988 ) ;
#125820=CIRCLE ( 'NONE', #61285, 0.06509327318403745899 ) ;
#125821=EDGE_LOOP ( 'NONE', ( #77116, #26298, #108913, #110127 ) ) ;
#125822=CARTESIAN_POINT ( 'NONE',  ( -6.050000000000018474, 2.500000000000000000, 2.611473670974873151 ) ) ;
#125823=EDGE_CURVE ( 'NONE', #54592, #42013, #128089, .T. ) ;
#125824=CONICAL_SURFACE ( 'NONE', #35960, 0.1000000000000002554, 0.003490658503988666988 ) ;
#125825=EDGE_CURVE ( 'NONE', #54921, #83172, #105079, .T. ) ;
#125826=ORIENTED_EDGE ( 'NONE', *, *, #123718, .F. ) ;
#125827=FACE_OUTER_BOUND ( 'NONE', #119403, .T. ) ;
#125828=DIRECTION ( 'NONE',  ( 0.000000000000000000, 0.000000000000000000, -1.000000000000000000 ) ) ;
#125829=ADVANCED_FACE ( 'NONE', ( #68594 ), #63337, .T. ) ;
#125830=CONICAL_SURFACE ( 'NONE', #113318, 0.09999999999999999167, 0.003490658503988666988 ) ;
#125831=ORIENTED_EDGE ( 'NONE', *, *, #36327, .F. ) ;
#125833=CARTESIAN_POINT ( 'NONE',  ( -2.100000000000034284, 2.500000000000000000, -4.230127018922201998 ) ) ;
#125834=CARTESIAN_POINT ( 'NONE',  ( -8.750000000000010658, 12.50000000000000000, 2.792790559304612064 ) ) ;
#125835=ADVANCED_FACE ( 'NONE', ( #28040 ), #58788, .T. ) ;
#125836=CARTESIAN_POINT ( 'NONE',  ( 1.449999999999951328, 2.500000000000000000, 2.411473670974873862 ) ) ;
#125837=DIRECTION ( 'NONE',  ( -0.000000000000000000, 1.000000000000000000, -0.000000000000000000 ) ) ;
#125838=ORIENTED_EDGE ( 'NONE', *, *, #14185, .T. ) ;
#125839=EDGE_CURVE ( 'NONE', #8618, #119760, #103031, .T. ) ;
#125840=EDGE_CURVE ( 'NONE', #41779, #104766, #90515, .T. ) ;
#125841=ADVANCED_FACE ( 'NONE', ( #90820 ), #123958, .T. ) ;
#125842=DIRECTION ( 'NONE',  ( 0.000000000000000000, 0.000000000000000000, 1.000000000000000000 ) ) ;
#125843=CARTESIAN_POINT ( 'NONE',  ( 8.149999999999923972, 2.500000000000000000, 2.511473670974873507 ) ) ;
#125844=ORIENTED_EDGE ( 'NONE', *, *, #109405, .T. ) ;
#125846=PLANE ( 'NONE',  #41361 ) ;
#125847=EDGE_CURVE ( 'NONE', #67678, #99722, #101292, .T. ) ;
#125848=DIRECTION ( 'NONE',  ( -4.274815082592931898E-19, -0.9999939076577903929, -0.003490651415223739937 ) ) ;
#125849=ORIENTED_EDGE ( 'NONE', *, *, #57353, .T. ) ;
#125851=CONICAL_SURFACE ( 'NONE', #69420, 0.1000000000000002554, 0.003490658503988666988 ) ;
#125852=AXIS2_PLACEMENT_3D ( 'NONE', #113240, #15676, #34053 ) ;
#125853=ORIENTED_EDGE ( 'NONE', *, *, #95058, .F. ) ;
#125854=CARTESIAN_POINT ( 'NONE',  ( 10.39999999999991331, 2.500000000000000000, -0.1000000000000023925 ) ) ;
#125855=DIRECTION ( 'NONE',  ( 0.000000000000000000, 0.000000000000000000, -1.000000000000000000 ) ) ;
#125856=DIRECTION ( 'NONE',  ( -0.000000000000000000, 1.000000000000000000, -0.000000000000000000 ) ) ;
#125857=ORIENTED_EDGE ( 'NONE', *, *, #72240, .T. ) ;
#125858=CARTESIAN_POINT ( 'NONE',  ( 7.899999999999924860, 12.50000000000000000, -4.395220292106239768 ) ) ;
#125859=AXIS2_PLACEMENT_3D ( 'NONE', #126964, #127606, #76574 ) ;
#125860=VECTOR ( 'NONE', #79901, 1000.000000000000000 ) ;
#125861=DIRECTION ( 'NONE',  ( 0.000000000000000000, -0.9999939076577903929, 0.003490651415223739937 ) ) ;
#125862=ORIENTED_EDGE ( 'NONE', *, *, #74665, .F. ) ;
#125863=CIRCLE ( 'NONE', #15031, 0.06509327318403745899 ) ;
#125864=VERTEX_POINT ( 'NONE', #111753 ) ;
#125865=CONICAL_SURFACE ( 'NONE', #4664, 0.1000000000000002554, 0.003490658503988666988 ) ;
#125866=DIRECTION ( 'NONE',  ( -0.000000000000000000, -1.000000000000000000, -0.000000000000000000 ) ) ;
#125867=VERTEX_POINT ( 'NONE', #112403 ) ;
#125868=FACE_OUTER_BOUND ( 'NONE', #94970, .T. ) ;
#125869=DIRECTION ( 'NONE',  ( 0.000000000000000000, 0.000000000000000000, 1.000000000000000000 ) ) ;
#125870=ORIENTED_EDGE ( 'NONE', *, *, #18016, .T. ) ;
#125871=DIRECTION ( 'NONE',  ( 0.000000000000000000, 0.000000000000000000, 1.000000000000000000 ) ) ;
#125872=LINE ( 'NONE', #106876, #2484 ) ;
#125873=ORIENTED_EDGE ( 'NONE', *, *, #16265, .F. ) ;
#125874=CARTESIAN_POINT ( 'NONE',  ( -9.800000000000004263, 2.500000000000000000, -0.3464101615137783474 ) ) ;
#125875=DIRECTION ( 'NONE',  ( -0.000000000000000000, 1.000000000000000000, -0.000000000000000000 ) ) ;
#125876=EDGE_CURVE ( 'NONE', #111738, #6241, #121815, .T. ) ;
#125877=CARTESIAN_POINT ( 'NONE',  ( 17.27572160909437926, -2.230096426605189031, -5.047229640871994327 ) ) ;
#125878=CARTESIAN_POINT ( 'NONE',  ( 0.3999999999999563904, 2.500000000000000000, 5.122947341949749323 ) ) ;
#125879=DIRECTION ( 'NONE',  ( -0.000000000000000000, 1.000000000000000000, -0.000000000000000000 ) ) ;
#125880=DIRECTION ( 'NONE',  ( 0.000000000000000000, 0.000000000000000000, 1.000000000000000000 ) ) ;
#125881=AXIS2_PLACEMENT_3D ( 'NONE', #86055, #116814, #75594 ) ;
#125883=ORIENTED_EDGE ( 'NONE', *, *, #39698, .F. ) ;
#125884=ORIENTED_EDGE ( 'NONE', *, *, #37823, .T. ) ;
#125885=ORIENTED_EDGE ( 'NONE', *, *, #97843, .F. ) ;
#125886=CARTESIAN_POINT ( 'NONE',  ( 5.599999999999931255, 12.50000000000000000, 4.741630453620009789 ) ) ;
#125887=LINE ( 'NONE', #68262, #115978 ) ;
#125888=CARTESIAN_POINT ( 'NONE',  ( -2.700000000000031264, 2.500000000000000000, 4.676537180435972552 ) ) ;
#125889=ORIENTED_EDGE ( 'NONE', *, *, #33380, .F. ) ;
#125890=EDGE_CURVE ( 'NONE', #5720, #25038, #65375, .T. ) ;
#125891=FACE_BOUND ( 'NONE', #92602, .T. ) ;
#125892=CIRCLE ( 'NONE', #100852, 0.1000000000000000472 ) ;
#125893=DIRECTION ( 'NONE',  ( -0.000000000000000000, -1.000000000000000000, -0.000000000000000000 ) ) ;
#125894=CARTESIAN_POINT ( 'NONE',  ( 2.899999999999945732, 2.500000000000000000, 0.09999999999999761857 ) ) ;
#125895=CONICAL_SURFACE ( 'NONE', #123841, 0.09999999999999999167, 0.003490658503988666988 ) ;
#125896=AXIS2_PLACEMENT_3D ( 'NONE', #93729, #43996, #32253 ) ;
#125897=DIRECTION ( 'NONE',  ( 0.000000000000000000, 0.000000000000000000, 1.000000000000000000 ) ) ;
#125898=VECTOR ( 'NONE', #129249, 1000.000000000000000 ) ;
#125899=PLANE ( 'NONE',  #107702 ) ;
#125900=FACE_OUTER_BOUND ( 'NONE', #100481, .T. ) ;
#125901=PLANE ( 'NONE',  #110278 ) ;
#125902=DIRECTION ( 'NONE',  ( 0.000000000000000000, 0.000000000000000000, -1.000000000000000000 ) ) ;
#125903=DIRECTION ( 'NONE',  ( 0.000000000000000000, 0.000000000000000000, 1.000000000000000000 ) ) ;
#125904=DIRECTION ( 'NONE',  ( 0.000000000000000000, 0.000000000000000000, 1.000000000000000000 ) ) ;
#125905=VECTOR ( 'NONE', #70969, 1000.000000000000000 ) ;
#125906=DIRECTION ( 'NONE',  ( 0.000000000000000000, 0.000000000000000000, 1.000000000000000000 ) ) ;
#125907=AXIS2_PLACEMENT_3D ( 'NONE', #13828, #114611, #112695 ) ;
#125908=VERTEX_POINT ( 'NONE', #89531 ) ;
#125909=ORIENTED_EDGE ( 'NONE', *, *, #90362, .T. ) ;
#125910=ORIENTED_EDGE ( 'NONE', *, *, #115309, .T. ) ;
#125911=AXIS2_PLACEMENT_3D ( 'NONE', #56868, #77178, #26150 ) ;
#125912=EDGE_LOOP ( 'NONE', ( #17369, #80688, #107749, #67847 ) ) ;
#125913=VECTOR ( 'NONE', #91669, 1000.000000000000000 ) ;
#125914=CARTESIAN_POINT ( 'NONE',  ( 3.349999999999942801, 2.500000000000000000, 2.757883832488649656 ) ) ;
#125915=ORIENTED_EDGE ( 'NONE', *, *, #88253, .F. ) ;
#125916=CARTESIAN_POINT ( 'NONE',  ( -10.65000000000000213, 2.500000000000000000, 6.941600689897073018 ) ) ;
#125917=EDGE_LOOP ( 'NONE', ( #95221, #48429, #25991, #5119 ) ) ;
#125918=ORIENTED_EDGE ( 'NONE', *, *, #115920, .T. ) ;
#125919=FACE_OUTER_BOUND ( 'NONE', #4174, .T. ) ;
#125921=CIRCLE ( 'NONE', #67410, 0.06509327318403745899 ) ;
#125922=CARTESIAN_POINT ( 'NONE',  ( 2.049999999999950084, 2.500000000000000000, -6.595190528383302109 ) ) ;
#125923=DIRECTION ( 'NONE',  ( 0.000000000000000000, 0.000000000000000000, 1.000000000000000000 ) ) ;
#125924=CARTESIAN_POINT ( 'NONE',  ( -1.700000000000034817, 2.500000000000000000, -4.230127018922201998 ) ) ;
#125925=CARTESIAN_POINT ( 'NONE',  ( -7.900000000000014566, 12.50000000000000000, -3.637306695894650055 ) ) ;
#125926=ORIENTED_EDGE ( 'NONE', *, *, #98371, .T. ) ;
#125927=EDGE_CURVE ( 'NONE', #114454, #67065, #113498, .T. ) ;
#125928=VERTEX_POINT ( 'NONE', #62664 ) ;
#125929=VERTEX_POINT ( 'NONE', #41102 ) ;
#125930=EDGE_LOOP ( 'NONE', ( #66184, #56915, #92486, #108526 ) ) ;
#125931=ADVANCED_FACE ( 'NONE', ( #22102 ), #31273, .T. ) ;
#125932=LINE ( 'NONE', #95208, #25331 ) ;
#125933=EDGE_CURVE ( 'NONE', #23542, #122530, #109298, .T. ) ;
#125934=EDGE_CURVE ( 'NONE', #87918, #104138, #61370, .T. ) ;
#125935=ORIENTED_EDGE ( 'NONE', *, *, #123008, .F. ) ;
#125936=EDGE_CURVE ( 'NONE', #117538, #80227, #126012, .T. ) ;
#125937=ADVANCED_FACE ( 'NONE', ( #80372 ), #102562, .T. ) ;
#125938=EDGE_LOOP ( 'NONE', ( #58581, #80940, #108242, #119575 ) ) ;
#125939=FACE_OUTER_BOUND ( 'NONE', #81084, .T. ) ;
#125940=LINE ( 'NONE', #95857, #49681 ) ;
#125941=CARTESIAN_POINT ( 'NONE',  ( -5.400000000000020783, 2.500000000000000000, 5.122947341949749323 ) ) ;
#125942=DIRECTION ( 'NONE',  ( 0.000000000000000000, 0.000000000000000000, 1.000000000000000000 ) ) ;
#125943=CONICAL_SURFACE ( 'NONE', #84177, 0.09999999999999999167, 0.003490658503988666988 ) ;
#125944=VECTOR ( 'NONE', #110978, 1000.000000000000000 ) ;
#125945=DIRECTION ( 'NONE',  ( -0.000000000000000000, 1.000000000000000000, -0.000000000000000000 ) ) ;
#125946=DIRECTION ( 'NONE',  ( 0.000000000000000000, 1.000000000000000000, 0.000000000000000000 ) ) ;
#125947=EDGE_CURVE ( 'NONE', #84422, #100878, #13135, .T. ) ;
#125948=ORIENTED_EDGE ( 'NONE', *, *, #61964, .F. ) ;
#125949=CARTESIAN_POINT ( 'NONE',  ( 12.69999999999989981, 12.50000000000000000, -0.3464101615137783474 ) ) ;
#125950=EDGE_CURVE ( 'NONE', #122396, #108909, #57061, .T. ) ;
#125951=VECTOR ( 'NONE', #28094, 1000.000000000000000 ) ;
#125952=EDGE_CURVE ( 'NONE', #107019, #20664, #46606, .T. ) ;
#125953=AXIS2_PLACEMENT_3D ( 'NONE', #33291, #52916, #73197 ) ;
#125954=EDGE_LOOP ( 'NONE', ( #87099, #21691 ) ) ;
#125956=ORIENTED_EDGE ( 'NONE', *, *, #8577, .F. ) ;
#125957=CARTESIAN_POINT ( 'NONE',  ( 0.4499999999999552136, 2.500000000000000000, 6.495190528383297135 ) ) ;
#125958=CARTESIAN_POINT ( 'NONE',  ( -0.6500000000000398792, 2.500000000000000000, -2.511473670974877948 ) ) ;
#125959=CIRCLE ( 'NONE', #23564, 0.1000000000000002554 ) ;
#125960=VERTEX_POINT ( 'NONE', #39810 ) ;
#125961=AXIS2_PLACEMENT_3D ( 'NONE', #84409, #64763, #26781 ) ;
#125962=DIRECTION ( 'NONE',  ( 0.000000000000000000, 0.000000000000000000, -1.000000000000000000 ) ) ;
#125963=CARTESIAN_POINT ( 'NONE',  ( -1.650000000000034772, 12.50000000000000000, 6.495190528383297135 ) ) ;
#125964=ORIENTED_EDGE ( 'NONE', *, *, #96390, .T. ) ;
#125965=AXIS2_PLACEMENT_3D ( 'NONE', #8287, #128079, #17454 ) ;
#125966=CARTESIAN_POINT ( 'NONE',  ( 9.599999999999914380, 2.500000000000000000, 3.737306695894644371 ) ) ;
#125967=VERTEX_POINT ( 'NONE', #119623 ) ;
#125968=ORIENTED_EDGE ( 'NONE', *, *, #1285, .F. ) ;
#125969=LINE ( 'NONE', #116150, #60388 ) ;
#125970=DIRECTION ( 'NONE',  ( 0.000000000000000000, 0.000000000000000000, 1.000000000000000000 ) ) ;
#125972=CARTESIAN_POINT ( 'NONE',  ( -1.450000000000035039, 2.500000000000000000, -2.611473670974877592 ) ) ;
#125973=AXIS2_PLACEMENT_3D ( 'NONE', #18636, #95912, #58584 ) ;
#125974=CARTESIAN_POINT ( 'NONE',  ( -8.950000000000004619, 12.50000000000000000, 6.148780366869520897 ) ) ;
#125975=DIRECTION ( 'NONE',  ( 0.000000000000000000, -0.9999939076577903929, 0.003490651415223739937 ) ) ;
#125976=AXIS2_PLACEMENT_3D ( 'NONE', #15884, #105567, #116665 ) ;
#125977=EDGE_LOOP ( 'NONE', ( #105072, #32689, #64989, #110388 ) ) ;
#125978=AXIS2_PLACEMENT_3D ( 'NONE', #106404, #86101, #36399 ) ;
#125979=DIRECTION ( 'NONE',  ( 0.000000000000000000, -0.9999939076577903929, 0.003490651415223739937 ) ) ;
#125980=VECTOR ( 'NONE', #62957, 1000.000000000000000 ) ;
#125981=ORIENTED_EDGE ( 'NONE', *, *, #95572, .F. ) ;
#125982=DIRECTION ( 'NONE',  ( -0.000000000000000000, -1.000000000000000000, -0.000000000000000000 ) ) ;
#125983=DIRECTION ( 'NONE',  ( -4.274815082592931898E-19, -0.9999939076577903929, -0.003490651415223739937 ) ) ;
#125984=ADVANCED_FACE ( 'NONE', ( #2415 ), #4726, .T. ) ;
#125985=CARTESIAN_POINT ( 'NONE',  ( -10.20000000000000639, 12.50000000000000000, -4.048810130592459089 ) ) ;
#125986=AXIS2_PLACEMENT_3D ( 'NONE', #53844, #114682, #74134 ) ;
#125987=ORIENTED_EDGE ( 'NONE', *, *, #98979, .T. ) ;
#125988=ADVANCED_FACE ( 'NONE', ( #44953 ), #38004, .T. ) ;
#125989=CONICAL_SURFACE ( 'NONE', #34075, 0.1000000000000000472, 0.003490658503988666988 ) ;
#125990=VECTOR ( 'NONE', #45364, 1000.000000000000000 ) ;
#125991=EDGE_CURVE ( 'NONE', #121009, #112979, #23349, .T. ) ;
#125992=DIRECTION ( 'NONE',  ( 0.000000000000000000, 0.000000000000000000, 1.000000000000000000 ) ) ;
#125993=LINE ( 'NONE', #106366, #78903 ) ;
#125994=AXIS2_PLACEMENT_3D ( 'NONE', #78561, #109283, #39298 ) ;
#125995=VERTEX_POINT ( 'NONE', #73118 ) ;
#125996=EDGE_CURVE ( 'NONE', #17997, #35493, #15468, .T. ) ;
#125997=CARTESIAN_POINT ( 'NONE',  ( 1.649999999999949729, 2.500000000000000000, 7.088010851410848190 ) ) ;
#125998=AXIS2_PLACEMENT_3D ( 'NONE', #47831, #38664, #87724 ) ;
#125999=VERTEX_POINT ( 'NONE', #95334 ) ;
#126000=CIRCLE ( 'NONE', #23611, 0.06509327318403745899 ) ;
#126001=CIRCLE ( 'NONE', #69580, 0.06509327318403745899 ) ;
#126002=VERTEX_POINT ( 'NONE', #43678 ) ;
#126003=AXIS2_PLACEMENT_3D ( 'NONE', #9864, #17730, #49804 ) ;
#126004=CARTESIAN_POINT ( 'NONE',  ( 7.499999999999923617, 2.500000000000000000, 0.6928203230275494784 ) ) ;
#126005=AXIS2_PLACEMENT_3D ( 'NONE', #86113, #16083, #95318 ) ;
#126006=VERTEX_POINT ( 'NONE', #52827 ) ;
#126007=CARTESIAN_POINT ( 'NONE',  ( 3.949999999999938005, 12.50000000000000000, 6.841600689897072485 ) ) ;
#126008=FACE_OUTER_BOUND ( 'NONE', #4319, .T. ) ;
#126009=DIRECTION ( 'NONE',  ( -0.000000000000000000, 1.000000000000000000, -0.000000000000000000 ) ) ;
#126010=ORIENTED_EDGE ( 'NONE', *, *, #79968, .T. ) ;
#126011=FACE_BOUND ( 'NONE', #103782, .T. ) ;
#126012=CIRCLE ( 'NONE', #107239, 0.06509327318403745899 ) ;
#126013=DIRECTION ( 'NONE',  ( -4.274815082592931898E-19, -0.9999939076577903929, -0.003490651415223739937 ) ) ;
#126014=ORIENTED_EDGE ( 'NONE', *, *, #63347, .T. ) ;
#126015=DIRECTION ( 'NONE',  ( 0.000000000000000000, 0.000000000000000000, 1.000000000000000000 ) ) ;
#126016=CARTESIAN_POINT ( 'NONE',  ( -11.64999999999999680, 12.50000000000000000, -6.430097255199260786 ) ) ;
#126017=EDGE_CURVE ( 'NONE', #108104, #29267, #54745, .T. ) ;
#126018=EDGE_LOOP ( 'NONE', ( #19237, #80734, #76240, #6582 ) ) ;
#126019=ORIENTED_EDGE ( 'NONE', *, *, #123684, .F. ) ;
#126020=ORIENTED_EDGE ( 'NONE', *, *, #82783, .F. ) ;
#126021=DIRECTION ( 'NONE',  ( -0.000000000000000000, 1.000000000000000000, -0.000000000000000000 ) ) ;
#126022=CARTESIAN_POINT ( 'NONE',  ( 5.599999999999934808, 12.50000000000000000, -4.676537180435978769 ) ) ;
#126023=FACE_OUTER_BOUND ( 'NONE', #56650, .T. ) ;
#126024=AXIS2_PLACEMENT_3D ( 'NONE', #104098, #54348, #56906 ) ;
#126025=FACE_BOUND ( 'NONE', #42430, .T. ) ;
#126026=VERTEX_POINT ( 'NONE', #114954 ) ;
#126028=FACE_OUTER_BOUND ( 'NONE', #18276, .T. ) ;
#126029=FACE_OUTER_BOUND ( 'NONE', #23088, .T. ) ;
#126030=CIRCLE ( 'NONE', #109615, 0.06509327318403745899 ) ;
#126031=FACE_OUTER_BOUND ( 'NONE', #53859, .T. ) ;
#126032=ADVANCED_FACE ( 'NONE', ( #82945 ), #124797, .T. ) ;
#126033=CONICAL_SURFACE ( 'NONE', #23640, 0.1000000000000000056, 0.003490658503988666988 ) ;
#126034=AXIS2_PLACEMENT_3D ( 'NONE', #88914, #108549, #128864 ) ;
#126035=FACE_OUTER_BOUND ( 'NONE', #840, .T. ) ;
#126036=AXIS2_PLACEMENT_3D ( 'NONE', #126633, #23922, #4246 ) ;
#126037=DIRECTION ( 'NONE',  ( 0.000000000000000000, 0.000000000000000000, -1.000000000000000000 ) ) ;
#126038=DIRECTION ( 'NONE',  ( 0.000000000000000000, 0.000000000000000000, -1.000000000000000000 ) ) ;
#126039=DIRECTION ( 'NONE',  ( 0.000000000000000000, 0.000000000000000000, 1.000000000000000000 ) ) ;
#126040=AXIS2_PLACEMENT_3D ( 'NONE', #70150, #78025, #19079 ) ;
#126041=AXIS2_PLACEMENT_3D ( 'NONE', #80936, #92679, #12804 ) ;
#126042=DIRECTION ( 'NONE',  ( 0.000000000000000000, 0.000000000000000000, -1.000000000000000000 ) ) ;
#126043=ORIENTED_EDGE ( 'NONE', *, *, #120029, .F. ) ;
#126044=VERTEX_POINT ( 'NONE', #115597 ) ;
#126045=EDGE_LOOP ( 'NONE', ( #76832, #6858 ) ) ;
#126046=ORIENTED_EDGE ( 'NONE', *, *, #55309, .F. ) ;
#126047=AXIS2_PLACEMENT_3D ( 'NONE', #33851, #112428, #12269 ) ;
#126048=ORIENTED_EDGE ( 'NONE', *, *, #122741, .F. ) ;
#126050=AXIS2_PLACEMENT_3D ( 'NONE', #29778, #80169, #59261 ) ;
#126051=DIRECTION ( 'NONE',  ( 0.000000000000000000, -0.000000000000000000, 1.000000000000000000 ) ) ;
#126052=VERTEX_POINT ( 'NONE', #85510 ) ;
#126053=EDGE_CURVE ( 'NONE', #11304, #54885, #3723, .T. ) ;
#126054=FACE_BOUND ( 'NONE', #32220, .T. ) ;
#126055=AXIS2_PLACEMENT_3D ( 'NONE', #19749, #91053, #9274 ) ;
#126056=CARTESIAN_POINT ( 'NONE',  ( -3.550000000000031797, 2.500000000000000000, -6.248780366869526759 ) ) ;
#126057=DIRECTION ( 'NONE',  ( -4.274815082592931898E-19, -0.9999939076577903929, -0.003490651415223739937 ) ) ;
#126058=FACE_OUTER_BOUND ( 'NONE', #33494, .T. ) ;
#126059=ADVANCED_FACE ( 'NONE', ( #124143 ), #21280, .T. ) ;
#126060=DIRECTION ( 'NONE',  ( 0.000000000000000000, 1.000000000000000000, 0.000000000000000000 ) ) ;
#126062=ORIENTED_EDGE ( 'NONE', *, *, #5363, .T. ) ;
#126063=CARTESIAN_POINT ( 'NONE',  ( -11.69999999999999574, 2.500000000000000000, 4.230127018922196669 ) ) ;
#126064=AXIS2_PLACEMENT_3D ( 'NONE', #53278, #93834, #63734 ) ;
#126065=ORIENTED_EDGE ( 'NONE', *, *, #66461, .F. ) ;
#126066=ORIENTED_EDGE ( 'NONE', *, *, #128975, .F. ) ;
#126067=VERTEX_POINT ( 'NONE', #125436 ) ;
#126068=DIRECTION ( 'NONE',  ( -0.000000000000000000, 1.000000000000000000, -0.000000000000000000 ) ) ;
#126069=CARTESIAN_POINT ( 'NONE',  ( 5.849999999999933031, 2.500000000000000000, -1.472243186433550122 ) ) ;
#126070=DIRECTION ( 'NONE',  ( 0.000000000000000000, 0.000000000000000000, -1.000000000000000000 ) ) ;
#126071=ORIENTED_EDGE ( 'NONE', *, *, #106607, .T. ) ;
#126072=CARTESIAN_POINT ( 'NONE',  ( 16.31259999906430025, 2.500000000000969891, -6.357732693023527837 ) ) ;
#126073=AXIS2_PLACEMENT_3D ( 'NONE', #45055, #73851, #84956 ) ;
#126074=AXIS2_PLACEMENT_3D ( 'NONE', #30454, #60560, #50712 ) ;
#126075=AXIS2_PLACEMENT_3D ( 'NONE', #19665, #68105, #20310 ) ;
#126076=DIRECTION ( 'NONE',  ( 0.000000000000000000, 1.000000000000000000, 0.000000000000000000 ) ) ;
#126077=ADVANCED_FACE ( 'NONE', ( #5644 ), #104500, .T. ) ;
#126078=DIRECTION ( 'NONE',  ( 0.000000000000000000, 0.000000000000000000, -1.000000000000000000 ) ) ;
#126080=CARTESIAN_POINT ( 'NONE',  ( -2.900000000000029665, 2.500000000000000000, 4.330127018922196314 ) ) ;
#126081=DIRECTION ( 'NONE',  ( 0.000000000000000000, 0.000000000000000000, -1.000000000000000000 ) ) ;
#126082=CIRCLE ( 'NONE', #69656, 0.06509327318403745899 ) ;
#126083=ORIENTED_EDGE ( 'NONE', *, *, #44553, .F. ) ;
#126084=DIRECTION ( 'NONE',  ( -0.000000000000000000, 1.000000000000000000, -0.000000000000000000 ) ) ;
#126085=AXIS2_PLACEMENT_3D ( 'NONE', #124845, #95382, #85557 ) ;
#126086=AXIS2_PLACEMENT_3D ( 'NONE', #15478, #32091, #111924 ) ;
#126087=EDGE_CURVE ( 'NONE', #100531, #15792, #81906, .T. ) ;
#126088=EDGE_LOOP ( 'NONE', ( #84123, #86742, #53911, #23662 ) ) ;
#126089=AXIS2_PLACEMENT_3D ( 'NONE', #82228, #22677, #10874 ) ;
#126090=ORIENTED_EDGE ( 'NONE', *, *, #111742, .T. ) ;
#126091=CARTESIAN_POINT ( 'NONE',  ( -4.400000000000028777, 2.500000000000000000, -3.883716857408426648 ) ) ;
#126092=ADVANCED_FACE ( 'NONE', ( #93402 ), #2487, .T. ) ;
#126093=DIRECTION ( 'NONE',  ( 0.000000000000000000, 0.000000000000000000, 1.000000000000000000 ) ) ;
#126094=DIRECTION ( 'NONE',  ( 0.000000000000000000, 1.000000000000000000, 0.000000000000000000 ) ) ;
#126095=EDGE_CURVE ( 'NONE', #91667, #52767, #102830, .T. ) ;
#126096=EDGE_CURVE ( 'NONE', #57274, #121670, #94721, .T. ) ;
#126097=EDGE_CURVE ( 'NONE', #98528, #49455, #31762, .T. ) ;
#126098=VERTEX_POINT ( 'NONE', #94043 ) ;
#126099=ORIENTED_EDGE ( 'NONE', *, *, #103635, .F. ) ;
#126101=CARTESIAN_POINT ( 'NONE',  ( 87.50000000000001421, 3.975344334345554120, -6.360552532166837914 ) ) ;
#126102=AXIS2_PLACEMENT_3D ( 'NONE', #10124, #99155, #58588 ) ;
#126103=CIRCLE ( 'NONE', #117767, 0.09999999999999982514 ) ;
#126104=AXIS2_PLACEMENT_3D ( 'NONE', #118362, #68615, #108550 ) ;
#126105=EDGE_CURVE ( 'NONE', #121644, #57128, #125820, .T. ) ;
#126106=LINE ( 'NONE', #113721, #75315 ) ;
#126107=EDGE_LOOP ( 'NONE', ( #113748, #120894 ) ) ;
#126108=VERTEX_POINT ( 'NONE', #84862 ) ;
#126109=EDGE_CURVE ( 'NONE', #119087, #127598, #4819, .T. ) ;
#126110=CARTESIAN_POINT ( 'NONE',  ( -10.84999999999999964, 2.500000000000000000, 1.372243186433545370 ) ) ;
#126111=CIRCLE ( 'NONE', #11180, 0.09999999999999982514 ) ;
#126112=EDGE_CURVE ( 'NONE', #88786, #71397, #54713, .T. ) ;
#126113=VERTEX_POINT ( 'NONE', #6280 ) ;
#126114=DIRECTION ( 'NONE',  ( 0.000000000000000000, 1.000000000000000000, 0.000000000000000000 ) ) ;
#126115=ADVANCED_FACE ( 'NONE', ( #126731 ), #97900, .T. ) ;
#126116=EDGE_CURVE ( 'NONE', #99549, #21005, #25764, .T. ) ;
#126117=DIRECTION ( 'NONE',  ( 0.000000000000000000, 0.000000000000000000, 1.000000000000000000 ) ) ;
#126118=ORIENTED_EDGE ( 'NONE', *, *, #83451, .F. ) ;
#126119=DIRECTION ( 'NONE',  ( -0.000000000000000000, -1.000000000000000000, -0.000000000000000000 ) ) ;
#126120=DIRECTION ( 'NONE',  ( 0.000000000000000000, -0.000000000000000000, 1.000000000000000000 ) ) ;
#126121=CARTESIAN_POINT ( 'NONE',  ( -1.250000000000037526, 2.500000000000000000, -1.372243186433550033 ) ) ;
#126122=DIRECTION ( 'NONE',  ( 0.000000000000000000, 0.000000000000000000, 1.000000000000000000 ) ) ;
#126123=EDGE_CURVE ( 'NONE', #57756, #72103, #14990, .T. ) ;
#126124=ORIENTED_EDGE ( 'NONE', *, *, #2682, .T. ) ;
#126125=LINE ( 'NONE', #64627, #50885 ) ;
#126126=CARTESIAN_POINT ( 'NONE',  ( -3.550000000000028244, 2.500000000000000000, -1.818653347947326138 ) ) ;
#126127=VERTEX_POINT ( 'NONE', #67800 ) ;
#126129=AXIS2_PLACEMENT_3D ( 'NONE', #115136, #16301, #15658 ) ;
#126130=CIRCLE ( 'NONE', #69695, 0.1000000000000002554 ) ;
#126131=CARTESIAN_POINT ( 'NONE',  ( -11.64999999999999858, 2.500000000000000000, -5.702370205355745902 ) ) ;
#126132=DIRECTION ( 'NONE',  ( 0.000000000000000000, 0.000000000000000000, -1.000000000000000000 ) ) ;
#126133=CARTESIAN_POINT ( 'NONE',  ( 6.449999999999930012, 2.500000000000000000, 1.818653347947321475 ) ) ;
#126134=CARTESIAN_POINT ( 'NONE',  ( 11.89999999999990798, 2.500000000000000000, -4.576537180435977348 ) ) ;
#126135=DIRECTION ( 'NONE',  ( 0.000000000000000000, 1.000000000000000000, 0.000000000000000000 ) ) ;
#126136=DIRECTION ( 'NONE',  ( 0.000000000000000000, 0.000000000000000000, 1.000000000000000000 ) ) ;
#126137=AXIS2_PLACEMENT_3D ( 'NONE', #13471, #92693, #3030 ) ;
#126138=VECTOR ( 'NONE', #45016, 1000.000000000000000 ) ;
#126139=DIRECTION ( 'NONE',  ( 0.000000000000000000, 0.000000000000000000, -1.000000000000000000 ) ) ;
#126140=AXIS2_PLACEMENT_3D ( 'NONE', #53621, #66012, #13679 ) ;
#126141=PLANE ( 'NONE',  #57389 ) ;
#126142=DIRECTION ( 'NONE',  ( 0.000000000000000000, 1.000000000000000000, 0.000000000000000000 ) ) ;
#126143=CIRCLE ( 'NONE', #128305, 0.1000000000000002554 ) ;
#126144=AXIS2_PLACEMENT_3D ( 'NONE', #115332, #125186, #6035 ) ;
#126145=DIRECTION ( 'NONE',  ( 0.000000000000000000, 0.000000000000000000, 1.000000000000000000 ) ) ;
#126146=EDGE_LOOP ( 'NONE', ( #116402, #42221, #64048, #92173 ) ) ;
#126147=AXIS2_PLACEMENT_3D ( 'NONE', #115857, #119090, #37319 ) ;
#126148=AXIS2_PLACEMENT_3D ( 'NONE', #59144, #99064, #49337 ) ;
#126149=AXIS2_PLACEMENT_3D ( 'NONE', #115392, #16558, #96411 ) ;
#126150=EDGE_LOOP ( 'NONE', ( #117837, #72696 ) ) ;
#126151=AXIS2_PLACEMENT_3D ( 'NONE', #50140, #58020, #89404 ) ;
#126152=FACE_OUTER_BOUND ( 'NONE', #123871, .T. ) ;
#126153=VECTOR ( 'NONE', #27585, 1000.000000000000000 ) ;
#126154=ORIENTED_EDGE ( 'NONE', *, *, #78886, .F. ) ;
#126155=CARTESIAN_POINT ( 'NONE',  ( -4.800000000000022915, 2.500000000000000000, 3.983716857408420076 ) ) ;
#126156=CARTESIAN_POINT ( 'NONE',  ( -3.750000000000027978, 12.50000000000000000, 7.122917578226811486 ) ) ;
#126157=DIRECTION ( 'NONE',  ( 0.000000000000000000, 0.000000000000000000, 1.000000000000000000 ) ) ;
#126158=ORIENTED_EDGE ( 'NONE', *, *, #103062, .T. ) ;
#126159=CARTESIAN_POINT ( 'NONE',  ( 17.50000000000000000, -2.500000000000000000, -2.922290670087884124 ) ) ;
#126160=EDGE_CURVE ( 'NONE', #65136, #9133, #107731, .T. ) ;
#126161=EDGE_CURVE ( 'NONE', #73855, #89818, #19209, .T. ) ;
#126162=DIRECTION ( 'NONE',  ( 0.000000000000000000, -0.9999939076577903929, 0.003490651415223739937 ) ) ;
#126163=CARTESIAN_POINT ( 'NONE',  ( -4.350000000000023626, 2.500000000000000000, 2.511473670974873507 ) ) ;
#126164=VERTEX_POINT ( 'NONE', #116884 ) ;
#126165=AXIS2_PLACEMENT_3D ( 'NONE', #4618, #121837, #82582 ) ;
#126166=DIRECTION ( 'NONE',  ( 0.000000000000000000, 0.000000000000000000, 1.000000000000000000 ) ) ;
#126167=EDGE_LOOP ( 'NONE', ( #24309, #100701 ) ) ;
#126168=ADVANCED_FACE ( 'NONE', ( #7582 ), #121921, .T. ) ;
#126169=EDGE_LOOP ( 'NONE', ( #34763, #57193 ) ) ;
#126170=ORIENTED_EDGE ( 'NONE', *, *, #43107, .F. ) ;
#126171=ORIENTED_EDGE ( 'NONE', *, *, #53836, .F. ) ;
#126172=FACE_OUTER_BOUND ( 'NONE', #14946, .T. ) ;
#126173=CARTESIAN_POINT ( 'NONE',  ( -7.499999999999980460, 12.50000000000000000, -2.276824562219559311E-15 ) ) ;
#126174=CIRCLE ( 'NONE', #688, 0.09999999999999999167 ) ;
#126175=FACE_OUTER_BOUND ( 'NONE', #115372, .T. ) ;
#126176=AXIS2_PLACEMENT_3D ( 'NONE', #100310, #100931, #2732 ) ;
#126177=DIRECTION ( 'NONE',  ( 0.000000000000000000, 0.000000000000000000, 1.000000000000000000 ) ) ;
#126179=EDGE_LOOP ( 'NONE', ( #77874, #120148 ) ) ;
#126180=CARTESIAN_POINT ( 'NONE',  ( 8.749999999999921840, 2.500000000000000000, -5.902370205355750521 ) ) ;
#126181=ORIENTED_EDGE ( 'NONE', *, *, #122381, .T. ) ;
#126182=LINE ( 'NONE', #75154, #124915 ) ;
#126183=CARTESIAN_POINT ( 'NONE',  ( -5.400000000000019895, 2.500000000000000000, 3.637306695894644726 ) ) ;
#126184=DIRECTION ( 'NONE',  ( 0.000000000000000000, 0.000000000000000000, 1.000000000000000000 ) ) ;
#126185=CARTESIAN_POINT ( 'NONE',  ( 20.06694580393955007, -2.635910463901628642, 2.269534205242087044 ) ) ;
#126186=VECTOR ( 'NONE', #3064, 1000.000000000000000 ) ;
#126187=AXIS2_PLACEMENT_3D ( 'NONE', #20693, #42271, #91355 ) ;
#126188=CIRCLE ( 'NONE', #128360, 0.06509327318403745899 ) ;
#126189=EDGE_LOOP ( 'NONE', ( #13894, #124060, #87254, #73092 ) ) ;
#126190=VECTOR ( 'NONE', #4925, 1000.000000000000000 ) ;
#126191=ORIENTED_EDGE ( 'NONE', *, *, #65947, .F. ) ;
#126192=ORIENTED_EDGE ( 'NONE', *, *, #18089, .T. ) ;
#126193=DIRECTION ( 'NONE',  ( 0.000000000000000000, -0.000000000000000000, 1.000000000000000000 ) ) ;
#126194=CARTESIAN_POINT ( 'NONE',  ( -8.550000000000014921, 12.50000000000000000, -6.213873640053559022 ) ) ;
#126195=FACE_OUTER_BOUND ( 'NONE', #63615, .T. ) ;
#126196=FACE_BOUND ( 'NONE', #15844, .T. ) ;
#126197=CONICAL_SURFACE ( 'NONE', #69762, 0.1000000000000002554, 0.003490658503988666988 ) ;
#126198=DIRECTION ( 'NONE',  ( 0.000000000000000000, 0.000000000000000000, 1.000000000000000000 ) ) ;
#126199=FACE_OUTER_BOUND ( 'NONE', #34008, .T. ) ;
#126200=DIRECTION ( 'NONE',  ( 0.000000000000000000, 0.000000000000000000, 1.000000000000000000 ) ) ;
#126201=CARTESIAN_POINT ( 'NONE',  ( -3.550000000000028244, 12.50000000000000000, -1.818653347947326138 ) ) ;
#126202=EDGE_CURVE ( 'NONE', #40952, #57912, #88453, .T. ) ;
#126203=AXIS2_PLACEMENT_3D ( 'NONE', #72909, #53285, #23155 ) ;
#126204=CONICAL_SURFACE ( 'NONE', #25860, 0.1000000000000002554, 0.003490658503988666988 ) ;
#126206=LINE ( 'NONE', #37195, #19579 ) ;
#126207=AXIS2_PLACEMENT_3D ( 'NONE', #52024, #122054, #82781 ) ;
#126208=CARTESIAN_POINT ( 'NONE',  ( -3.350000000000028955, 2.500000000000000000, 5.802370205355744659 ) ) ;
#126209=AXIS2_PLACEMENT_3D ( 'NONE', #46685, #108807, #38830 ) ;
#126210=CARTESIAN_POINT ( 'NONE',  ( 8.949999999999921130, 2.500000000000000000, 1.818653347947321475 ) ) ;
#126211=ORIENTED_EDGE ( 'NONE', *, *, #46315, .F. ) ;
#126212=ORIENTED_EDGE ( 'NONE', *, *, #4, .F. ) ;
#126213=EDGE_LOOP ( 'NONE', ( #67943, #89838, #101368, #68786 ) ) ;
#126214=ORIENTED_EDGE ( 'NONE', *, *, #124463, .T. ) ;
#126215=EDGE_CURVE ( 'NONE', #5786, #121359, #65467, .T. ) ;
#126216=DIRECTION ( 'NONE',  ( 0.000000000000000000, 0.000000000000000000, 1.000000000000000000 ) ) ;
#126218=FACE_BOUND ( 'NONE', #45102, .T. ) ;
#126219=CARTESIAN_POINT ( 'NONE',  ( 2.299999999999949640, 2.500000000000000000, -4.776537180435977525 ) ) ;
#126221=AXIS2_PLACEMENT_3D ( 'NONE', #31323, #72530, #111122 ) ;
#126222=VERTEX_POINT ( 'NONE', #36434 ) ;
#126223=FACE_OUTER_BOUND ( 'NONE', #43493, .T. ) ;
#126224=VECTOR ( 'NONE', #115770, 1000.000000000000000 ) ;
#126225=EDGE_CURVE ( 'NONE', #7522, #108949, #21570, .T. ) ;
#126227=ORIENTED_EDGE ( 'NONE', *, *, #16843, .T. ) ;
#126228=DIRECTION ( 'NONE',  ( -0.000000000000000000, -1.000000000000000000, -0.000000000000000000 ) ) ;
#126229=CARTESIAN_POINT ( 'NONE',  ( 5.599999999999933031, 2.500000000000000000, 0.4464101615137735513 ) ) ;
#126230=VECTOR ( 'NONE', #29751, 1000.000000000000000 ) ;
#126231=AXIS2_PLACEMENT_3D ( 'NONE', #100540, #29878, #1055 ) ;
#126232=AXIS2_PLACEMENT_3D ( 'NONE', #21420, #86719, #118753 ) ;
#126233=VECTOR ( 'NONE', #102448, 1000.000000000000000 ) ;
#126234=VECTOR ( 'NONE', #78009, 1000.000000000000000 ) ;
#126235=ORIENTED_EDGE ( 'NONE', *, *, #46908, .F. ) ;
#126236=CARTESIAN_POINT ( 'NONE',  ( -11.44999999999999751, 2.500000000000000000, 2.611473670974873151 ) ) ;
#126237=CARTESIAN_POINT ( 'NONE',  ( 0.3999999999999555023, 12.50000000000000000, 4.330127018922196314 ) ) ;
#126238=AXIS2_PLACEMENT_3D ( 'NONE', #86350, #74613, #35978 ) ;
#126239=EDGE_LOOP ( 'NONE', ( #121766, #72502 ) ) ;
#126240=VECTOR ( 'NONE', #119284, 1000.000000000000000 ) ;
#126241=DIRECTION ( 'NONE',  ( -0.000000000000000000, -1.000000000000000000, -0.000000000000000000 ) ) ;
#126242=FACE_OUTER_BOUND ( 'NONE', #8176, .T. ) ;
#126243=VERTEX_POINT ( 'NONE', #87433 ) ;
#126244=DIRECTION ( 'NONE',  ( -0.000000000000000000, 1.000000000000000000, -0.000000000000000000 ) ) ;
#126245=AXIS2_PLACEMENT_3D ( 'NONE', #91683, #110669, #51133 ) ;
#126246=ORIENTED_EDGE ( 'NONE', *, *, #111164, .T. ) ;
#126247=EDGE_LOOP ( 'NONE', ( #1090, #7880, #126942, #103847 ) ) ;
#126248=DIRECTION ( 'NONE',  ( 0.000000000000000000, 1.000000000000000000, 0.000000000000000000 ) ) ;
#126249=ORIENTED_EDGE ( 'NONE', *, *, #15606, .T. ) ;
#126250=CARTESIAN_POINT ( 'NONE',  ( -4.150000000000024336, 2.500000000000000000, -2.165063509461101710 ) ) ;
#126251=CARTESIAN_POINT ( 'NONE',  ( 13.34999999999990017, 12.50000000000000000, 2.792790559304612064 ) ) ;
#126252=EDGE_CURVE ( 'NONE', #36118, #7221, #65170, .T. ) ;
#126253=ORIENTED_EDGE ( 'NONE', *, *, #51344, .F. ) ;
#126254=DIRECTION ( 'NONE',  ( 0.000000000000000000, 0.000000000000000000, 1.000000000000000000 ) ) ;
#126255=DIRECTION ( 'NONE',  ( 0.000000000000000000, 0.000000000000000000, 1.000000000000000000 ) ) ;
#126256=CARTESIAN_POINT ( 'NONE',  ( 7.499999999999961808, 12.50000000000000000, -4.330127018922201643 ) ) ;
#126258=CARTESIAN_POINT ( 'NONE',  ( -0.8500000000000382805, 12.50000000000000000, -2.922977105672691422 ) ) ;
#126259=CARTESIAN_POINT ( 'NONE',  ( -1.650000000000034772, 12.50000000000000000, 2.165063509461097713 ) ) ;
#126260=EDGE_CURVE ( 'NONE', #38409, #6262, #16741, .T. ) ;
#126262=EDGE_CURVE ( 'NONE', #14356, #27444, #46885, .T. ) ;
#126263=AXIS2_PLACEMENT_3D ( 'NONE', #68718, #59585, #9806 ) ;
#126264=ORIENTED_EDGE ( 'NONE', *, *, #95996, .F. ) ;
#126265=EDGE_LOOP ( 'NONE', ( #49017, #110859, #80902, #18394 ) ) ;
#126266=CARTESIAN_POINT ( 'NONE',  ( 5.649999999999934630, 12.50000000000000000, -2.576566944158915184 ) ) ;
#126267=DIRECTION ( 'NONE',  ( -0.000000000000000000, -1.000000000000000000, -0.000000000000000000 ) ) ;
#126268=ADVANCED_FACE ( 'NONE', ( #77611 ), #108369, .T. ) ;
#126269=DIRECTION ( 'NONE',  ( -0.000000000000000000, -1.000000000000000000, -0.000000000000000000 ) ) ;
#126270=ORIENTED_EDGE ( 'NONE', *, *, #69046, .F. ) ;
#126271=VERTEX_POINT ( 'NONE', #8863 ) ;
#126272=EDGE_CURVE ( 'NONE', #113921, #99720, #9030, .T. ) ;
#126273=ORIENTED_EDGE ( 'NONE', *, *, #2756, .T. ) ;
#126274=EDGE_CURVE ( 'NONE', #105841, #9122, #111438, .T. ) ;
#126275=DIRECTION ( 'NONE',  ( -0.000000000000000000, 1.000000000000000000, -0.000000000000000000 ) ) ;
#126276=AXIS2_PLACEMENT_3D ( 'NONE', #104789, #113993, #3385 ) ;
#126278=CONICAL_SURFACE ( 'NONE', #30142, 0.09999999999999982514, 0.003490658503988666988 ) ;
#126279=DIRECTION ( 'NONE',  ( 0.000000000000000000, 0.000000000000000000, 1.000000000000000000 ) ) ;
#126281=EDGE_CURVE ( 'NONE', #108388, #107957, #63142, .T. ) ;
#126282=CARTESIAN_POINT ( 'NONE',  ( -14.14999999999998614, 2.500000000000000000, -2.857883832488651521 ) ) ;
#126283=DIRECTION ( 'NONE',  ( 0.000000000000000000, 0.000000000000000000, -1.000000000000000000 ) ) ;
#126285=DIRECTION ( 'NONE',  ( 0.000000000000000000, 0.000000000000000000, 1.000000000000000000 ) ) ;
#126286=CARTESIAN_POINT ( 'NONE',  ( 11.64999999999990443, 2.500000000000000000, -7.088010851410853519 ) ) ;
#126287=VECTOR ( 'NONE', #75645, 1000.000000000000000 ) ;
#126288=CARTESIAN_POINT ( 'NONE',  ( -0.2000000000000339284, 12.50000000000000000, -0.3464101615137759604 ) ) ;
#126289=EDGE_CURVE ( 'NONE', #41760, #69690, #95976, .T. ) ;
#126290=ORIENTED_EDGE ( 'NONE', *, *, #43879, .F. ) ;
#126291=CONICAL_SURFACE ( 'NONE', #69757, 0.09999999999999982514, 0.003490658503988666988 ) ;
#126292=CARTESIAN_POINT ( 'NONE',  ( 5.799999999999933209, 2.500000000000000000, -2.385244779468109755E-15 ) ) ;
#126293=ORIENTED_EDGE ( 'NONE', *, *, #90511, .T. ) ;
#126294=VERTEX_POINT ( 'NONE', #123818 ) ;
#126295=FACE_OUTER_BOUND ( 'NONE', #104441, .T. ) ;
#126296=LINE ( 'NONE', #5212, #36377 ) ;
#126297=PLANE ( 'NONE',  #80092 ) ;
#126298=DIRECTION ( 'NONE',  ( -0.000000000000000000, -1.000000000000000000, -0.000000000000000000 ) ) ;
#126300=CIRCLE ( 'NONE', #53138, 0.09999999999999982514 ) ;
#126301=PLANE ( 'NONE',  #59543 ) ;
#126302=AXIS2_PLACEMENT_3D ( 'NONE', #83101, #32076, #123020 ) ;
#126303=AXIS2_PLACEMENT_3D ( 'NONE', #118626, #37512, #28979 ) ;
#126304=DIRECTION ( 'NONE',  ( 0.000000000000000000, 0.000000000000000000, 1.000000000000000000 ) ) ;
#126305=ORIENTED_EDGE ( 'NONE', *, *, #8570, .F. ) ;
#126306=CARTESIAN_POINT ( 'NONE',  ( 0.8499999999999557909, 2.500000000000000000, -7.188010851410854052 ) ) ;
#126307=AXIS2_PLACEMENT_3D ( 'NONE', #66965, #77450, #68263 ) ;
#126308=AXIS2_PLACEMENT_3D ( 'NONE', #66470, #35733, #114285 ) ;
#126310=ORIENTED_EDGE ( 'NONE', *, *, #83296, .F. ) ;
#126311=ORIENTED_EDGE ( 'NONE', *, *, #77752, .F. ) ;
#126312=VERTEX_POINT ( 'NONE', #23706 ) ;
#126313=VERTEX_POINT ( 'NONE', #21783 ) ;
#126314=DIRECTION ( 'NONE',  ( 0.000000000000000000, -0.000000000000000000, 1.000000000000000000 ) ) ;
#126315=DIRECTION ( 'NONE',  ( -0.000000000000000000, 1.000000000000000000, -0.000000000000000000 ) ) ;
#126316=EDGE_LOOP ( 'NONE', ( #111626, #102442 ) ) ;
#126317=DIRECTION ( 'NONE',  ( 0.000000000000000000, -0.000000000000000000, 1.000000000000000000 ) ) ;
#126318=EDGE_CURVE ( 'NONE', #128359, #71554, #1472, .T. ) ;
#126319=CARTESIAN_POINT ( 'NONE',  ( 2.500000000000002220, 0.9166666666666682950, -9.999999999999998224 ) ) ;
#126320=VECTOR ( 'NONE', #47746, 1000.000000000000000 ) ;
#126321=AXIS2_PLACEMENT_3D ( 'NONE', #73176, #12312, #102621 ) ;
#126322=CARTESIAN_POINT ( 'NONE',  ( -0.8500000000000386136, 12.50000000000000000, 1.472243186433545459 ) ) ;
#126323=ORIENTED_EDGE ( 'NONE', *, *, #14812, .T. ) ;
#126324=CIRCLE ( 'NONE', #40665, 0.06509327318403745899 ) ;
#126325=CIRCLE ( 'NONE', #88663, 0.9999999999999998890 ) ;
#126326=DIRECTION ( 'NONE',  ( -0.000000000000000000, -1.000000000000000000, -0.000000000000000000 ) ) ;
#126327=DIRECTION ( 'NONE',  ( 0.000000000000000000, 0.000000000000000000, -1.000000000000000000 ) ) ;
#126328=EDGE_CURVE ( 'NONE', #63386, #31251, #15278, .T. ) ;
#126329=ORIENTED_EDGE ( 'NONE', *, *, #70900, .T. ) ;
#126330=CONICAL_SURFACE ( 'NONE', #69893, 0.09999999999999999167, 0.003490658503988666988 ) ;
#126331=AXIS2_PLACEMENT_3D ( 'NONE', #73159, #103268, #113069 ) ;
#126332=VECTOR ( 'NONE', #12128, 1000.000000000000000 ) ;
#126333=ORIENTED_EDGE ( 'NONE', *, *, #109684, .T. ) ;
#126334=VERTEX_POINT ( 'NONE', #51253 ) ;
#126335=DIRECTION ( 'NONE',  ( -0.000000000000000000, -1.000000000000000000, -0.000000000000000000 ) ) ;
#126336=CARTESIAN_POINT ( 'NONE',  ( -4.800000000000026468, 12.50000000000000000, -4.676537180435978769 ) ) ;
#126337=AXIS2_PLACEMENT_3D ( 'NONE', #20092, #72418, #90094 ) ;
#126338=VECTOR ( 'NONE', #20208, 1000.000000000000000 ) ;
#126339=AXIS2_PLACEMENT_3D ( 'NONE', #47839, #18357, #17701 ) ;
#126340=CIRCLE ( 'NONE', #80284, 0.06509327318403745899 ) ;
#126341=VERTEX_POINT ( 'NONE', #23060 ) ;
#126342=CARTESIAN_POINT ( 'NONE',  ( -4.350000000000023626, 2.500000000000000000, 1.818653347947321475 ) ) ;
#126343=DIRECTION ( 'NONE',  ( 0.000000000000000000, -0.9999939076577903929, 0.003490651415223739937 ) ) ;
#126345=LINE ( 'NONE', #76593, #23221 ) ;
#126346=ORIENTED_EDGE ( 'NONE', *, *, #27051, .F. ) ;
#126347=CARTESIAN_POINT ( 'NONE',  ( -6.450000000000017941, 2.500000000000000000, -2.511473670974877948 ) ) ;
#126348=ORIENTED_EDGE ( 'NONE', *, *, #61581, .F. ) ;
#126349=EDGE_LOOP ( 'NONE', ( #78107, #114139 ) ) ;
#126350=ORIENTED_EDGE ( 'NONE', *, *, #91674, .F. ) ;
#126351=CARTESIAN_POINT ( 'NONE',  ( 2.099999999999950351, 12.50000000000000000, -0.7579135962115916003 ) ) ;
#126352=FACE_BOUND ( 'NONE', #122442, .T. ) ;
#126353=FACE_OUTER_BOUND ( 'NONE', #10486, .T. ) ;
#126354=AXIS2_PLACEMENT_3D ( 'NONE', #90063, #50806, #80268 ) ;
#126355=DIRECTION ( 'NONE',  ( -0.000000000000000000, 1.000000000000000000, -0.000000000000000000 ) ) ;
#126356=DIRECTION ( 'NONE',  ( 0.000000000000000000, 1.000000000000000000, 0.000000000000000000 ) ) ;
#126357=ADVANCED_FACE ( 'NONE', ( #82636 ), #32899, .T. ) ;
#126358=VERTEX_POINT ( 'NONE', #93735 ) ;
#126360=DIRECTION ( 'NONE',  ( 0.000000000000000000, 0.000000000000000000, -1.000000000000000000 ) ) ;
#126361=DIRECTION ( 'NONE',  ( 0.000000000000000000, 0.000000000000000000, -1.000000000000000000 ) ) ;
#126362=FACE_OUTER_BOUND ( 'NONE', #60990, .T. ) ;
#126363=ORIENTED_EDGE ( 'NONE', *, *, #80016, .T. ) ;
#126364=CIRCLE ( 'NONE', #30242, 7.500000000000000000 ) ;
#126365=EDGE_CURVE ( 'NONE', #61083, #2989, #112737, .T. ) ;
#126366=AXIS2_PLACEMENT_3D ( 'NONE', #1910, #52964, #54248 ) ;
#126367=LINE ( 'NONE', #36709, #36429 ) ;
#126368=DIRECTION ( 'NONE',  ( 0.000000000000000000, 0.000000000000000000, 1.000000000000000000 ) ) ;
#126369=ORIENTED_EDGE ( 'NONE', *, *, #342, .F. ) ;
#126370=EDGE_CURVE ( 'NONE', #67997, #29869, #71436, .T. ) ;
#126371=PLANE ( 'NONE',  #114996 ) ;
#126372=DIRECTION ( 'NONE',  ( 0.000000000000000000, 0.000000000000000000, 1.000000000000000000 ) ) ;
#126373=EDGE_CURVE ( 'NONE', #59250, #89734, #121713, .T. ) ;
#126374=FACE_BOUND ( 'NONE', #120449, .T. ) ;
#126375=DIRECTION ( 'NONE',  ( 0.000000000000000000, 0.000000000000000000, -1.000000000000000000 ) ) ;
#126376=CONICAL_SURFACE ( 'NONE', #38575, 0.09999999999999982514, 0.003490658503988666988 ) ;
#126377=ORIENTED_EDGE ( 'NONE', *, *, #17170, .T. ) ;
#126378=CARTESIAN_POINT ( 'NONE',  ( -0.6500000000000403233, 2.500000000000000000, 6.148780366869520009 ) ) ;
#126379=DIRECTION ( 'NONE',  ( 0.000000000000000000, 0.000000000000000000, -1.000000000000000000 ) ) ;
#126380=EDGE_CURVE ( 'NONE', #56480, #110736, #11297, .T. ) ;
#126381=VERTEX_POINT ( 'NONE', #72810 ) ;
#126382=ORIENTED_EDGE ( 'NONE', *, *, #120544, .F. ) ;
#126383=EDGE_CURVE ( 'NONE', #13274, #30016, #94528, .T. ) ;
#126385=VERTEX_POINT ( 'NONE', #12578 ) ;
#126386=CARTESIAN_POINT ( 'NONE',  ( 11.84999999999990727, 12.50000000000000000, -2.511473670974877948 ) ) ;
#126387=FACE_OUTER_BOUND ( 'NONE', #92309, .T. ) ;
#126388=AXIS2_PLACEMENT_3D ( 'NONE', #119761, #51684, #30119 ) ;
#126389=VECTOR ( 'NONE', #51196, 1000.000000000000000 ) ;
#126390=DIRECTION ( 'NONE',  ( 0.000000000000000000, 0.000000000000000000, 1.000000000000000000 ) ) ;
#126391=AXIS2_PLACEMENT_3D ( 'NONE', #36086, #114631, #26271 ) ;
#126392=DIRECTION ( 'NONE',  ( 0.000000000000000000, -0.000000000000000000, 1.000000000000000000 ) ) ;
#126393=CIRCLE ( 'NONE', #40738, 0.1000000000000002554 ) ;
#126394=ORIENTED_EDGE ( 'NONE', *, *, #78037, .F. ) ;
#126395=CARTESIAN_POINT ( 'NONE',  ( -10.40000000000000213, 2.500000000000000000, 4.430127018922196847 ) ) ;
#126396=DIRECTION ( 'NONE',  ( 0.000000000000000000, 1.000000000000000000, 0.000000000000000000 ) ) ;
#126397=CARTESIAN_POINT ( 'NONE',  ( -6.650000000000014566, 12.50000000000000000, 1.472243186433545459 ) ) ;
#126398=DIRECTION ( 'NONE',  ( -4.274815082592931898E-19, -0.9999939076577903929, -0.003490651415223739937 ) ) ;
#126399=ORIENTED_EDGE ( 'NONE', *, *, #17496, .T. ) ;
#126400=DIRECTION ( 'NONE',  ( 0.000000000000000000, -0.000000000000000000, 1.000000000000000000 ) ) ;
#126402=DIRECTION ( 'NONE',  ( 0.000000000000000000, 0.000000000000000000, -1.000000000000000000 ) ) ;
#126403=CARTESIAN_POINT ( 'NONE',  ( 11.89999999999990443, 12.50000000000000000, -0.3464101615137782364 ) ) ;
#126404=ORIENTED_EDGE ( 'NONE', *, *, #58885, .F. ) ;
#126405=DIRECTION ( 'NONE',  ( 0.000000000000000000, 1.000000000000000000, 0.000000000000000000 ) ) ;
#126406=CARTESIAN_POINT ( 'NONE',  ( 17.50000000000000000, -2.499999999999999556, -3.666666666666664298 ) ) ;
#126407=EDGE_CURVE ( 'NONE', #44421, #8315, #75745, .T. ) ;
#126408=DIRECTION ( 'NONE',  ( -0.000000000000000000, -1.000000000000000000, -0.000000000000000000 ) ) ;
#126409=CONICAL_SURFACE ( 'NONE', #113896, 0.09999999999999999167, 0.003490658503988666988 ) ;
#126410=DIRECTION ( 'NONE',  ( 0.000000000000000000, 0.000000000000000000, 1.000000000000000000 ) ) ;
#126411=EDGE_LOOP ( 'NONE', ( #116229, #81871 ) ) ;
#126412=AXIS2_PLACEMENT_3D ( 'NONE', #82200, #54028, #33738 ) ;
#126413=DIRECTION ( 'NONE',  ( 0.000000000000000000, 0.000000000000000000, -1.000000000000000000 ) ) ;
#126414=CARTESIAN_POINT ( 'NONE',  ( -6.650000000000019007, 12.50000000000000000, -5.802370205355749988 ) ) ;
#126415=CONICAL_SURFACE ( 'NONE', #30284, 0.1000000000000002554, 0.003490658503988666988 ) ;
#126418=FACE_OUTER_BOUND ( 'NONE', #36582, .T. ) ;
#126419=CARTESIAN_POINT ( 'NONE',  ( 10.39999999999991509, 2.500000000000000000, -0.7928203230275543412 ) ) ;
#126420=EDGE_CURVE ( 'NONE', #43475, #99497, #111419, .T. ) ;
#126421=CONICAL_SURFACE ( 'NONE', #111848, 0.09999999999999999167, 0.003490658503988666988 ) ;
#126422=VERTEX_POINT ( 'NONE', #101631 ) ;
#126423=AXIS2_PLACEMENT_3D ( 'NONE', #105964, #96137, #24827 ) ;
#126424=ORIENTED_EDGE ( 'NONE', *, *, #46174, .T. ) ;
#126425=CIRCLE ( 'NONE', #13534, 0.1000000000000000056 ) ;
#126426=LINE ( 'NONE', #45294, #99321 ) ;
#126427=ORIENTED_EDGE ( 'NONE', *, *, #15445, .F. ) ;
#126428=DIRECTION ( 'NONE',  ( 0.000000000000000000, 0.000000000000000000, 1.000000000000000000 ) ) ;
#126429=ADVANCED_FACE ( 'NONE', ( #51884 ), #90307, .T. ) ;
#126430=CIRCLE ( 'NONE', #59647, 0.06509327318403745899 ) ;
#126431=VERTEX_POINT ( 'NONE', #2114 ) ;
#126432=EDGE_LOOP ( 'NONE', ( #128202, #71915 ) ) ;
#126433=VERTEX_POINT ( 'NONE', #83278 ) ;
#126434=EDGE_CURVE ( 'NONE', #9737, #104138, #23512, .T. ) ;
#126436=EDGE_CURVE ( 'NONE', #86367, #11533, #98723, .T. ) ;
#126437=CIRCLE ( 'NONE', #47018, 0.1000000000000002554 ) ;
#126438=CARTESIAN_POINT ( 'NONE',  ( -6.900000000000019007, 2.500000000000000000, -0.3464101615137783474 ) ) ;
#126439=AXIS2_PLACEMENT_3D ( 'NONE', #27362, #80201, #87580 ) ;
#126441=EDGE_CURVE ( 'NONE', #34192, #29616, #102941, .T. ) ;
#126442=DIRECTION ( 'NONE',  ( 0.000000000000000000, 0.000000000000000000, 1.000000000000000000 ) ) ;
#126443=DIRECTION ( 'NONE',  ( 0.000000000000000000, -0.9999939076577903929, 0.003490651415223739937 ) ) ;
#126444=CIRCLE ( 'NONE', #30308, 0.09999999999999982514 ) ;
#126445=DIRECTION ( 'NONE',  ( 0.000000000000000000, 1.000000000000000000, 0.000000000000000000 ) ) ;
#126446=ORIENTED_EDGE ( 'NONE', *, *, #13020, .F. ) ;
#126447=CARTESIAN_POINT ( 'NONE',  ( 1.899999999999951283, 12.50000000000000000, -3.983716857408426293 ) ) ;
#126448=ADVANCED_FACE ( 'NONE', ( #72172 ), #88248, .T. ) ;
#126449=ORIENTED_EDGE ( 'NONE', *, *, #53733, .T. ) ;
#126450=ADVANCED_FACE ( 'NONE', ( #83898 ), #96568, .T. ) ;
#126451=EDGE_LOOP ( 'NONE', ( #117892, #20403, #79853, #99678 ) ) ;
#126453=ORIENTED_EDGE ( 'NONE', *, *, #110931, .F. ) ;
#126454=CARTESIAN_POINT ( 'NONE',  ( -8.150000000000009237, 12.50000000000000000, 6.213873640053558134 ) ) ;
#126455=VERTEX_POINT ( 'NONE', #4675 ) ;
#126456=ORIENTED_EDGE ( 'NONE', *, *, #87514, .T. ) ;
#126457=AXIS2_PLACEMENT_3D ( 'NONE', #88551, #100943, #58475 ) ;
#126458=CARTESIAN_POINT ( 'NONE',  ( -13.14999999999999147, 12.50000000000000000, 2.511473670974877503 ) ) ;
#126459=DIRECTION ( 'NONE',  ( 0.000000000000000000, 0.000000000000000000, 1.000000000000000000 ) ) ;
#126460=DIRECTION ( 'NONE',  ( 0.000000000000000000, -0.000000000000000000, 1.000000000000000000 ) ) ;
#126461=DIRECTION ( 'NONE',  ( 0.000000000000000000, 1.000000000000000000, 0.000000000000000000 ) ) ;
#126462=DIRECTION ( 'NONE',  ( -0.000000000000000000, -1.000000000000000000, -0.000000000000000000 ) ) ;
#126463=EDGE_LOOP ( 'NONE', ( #127282, #71311 ) ) ;
#126464=DIRECTION ( 'NONE',  ( 0.000000000000000000, 0.000000000000000000, -1.000000000000000000 ) ) ;
#126465=CIRCLE ( 'NONE', #72188, 0.06509327318403745899 ) ;
#126466=VECTOR ( 'NONE', #78421, 1000.000000000000000 ) ;
#126468=DIRECTION ( 'NONE',  ( 0.000000000000000000, 0.000000000000000000, 1.000000000000000000 ) ) ;
#126469=ORIENTED_EDGE ( 'NONE', *, *, #91837, .T. ) ;
#126470=DIRECTION ( 'NONE',  ( -4.274815082592931898E-19, -0.9999939076577903929, -0.003490651415223739937 ) ) ;
#126471=ORIENTED_EDGE ( 'NONE', *, *, #52939, .F. ) ;
#126472=ORIENTED_EDGE ( 'NONE', *, *, #115591, .T. ) ;
#126473=CARTESIAN_POINT ( 'NONE',  ( 8.749999999999957367, 2.500000000000000000, -6.495190528383302464 ) ) ;
#126474=DIRECTION ( 'NONE',  ( -0.000000000000000000, -1.000000000000000000, -0.000000000000000000 ) ) ;
#126475=CARTESIAN_POINT ( 'NONE',  ( -13.34999999999999076, 2.500000000000000000, 2.957883832488652942 ) ) ;
#126476=ADVANCED_FACE ( 'NONE', ( #45934 ), #57010, .T. ) ;
#126477=DIRECTION ( 'NONE',  ( -0.000000000000000000, -1.000000000000000000, -0.000000000000000000 ) ) ;
#126478=CIRCLE ( 'NONE', #5266, 0.1000000000000002554 ) ;
#126479=DIRECTION ( 'NONE',  ( 0.000000000000000000, -0.9999939076577903929, 0.003490651415223739937 ) ) ;
#126480=ORIENTED_EDGE ( 'NONE', *, *, #98655, .T. ) ;
#126481=FACE_OUTER_BOUND ( 'NONE', #105931, .T. ) ;
#126482=DIRECTION ( 'NONE',  ( 0.000000000000000000, 0.000000000000000000, 1.000000000000000000 ) ) ;
#126483=DIRECTION ( 'NONE',  ( 0.000000000000000000, 0.000000000000000000, -1.000000000000000000 ) ) ;
#126484=FACE_OUTER_BOUND ( 'NONE', #115028, .T. ) ;
#126485=DIRECTION ( 'NONE',  ( -0.000000000000000000, 1.000000000000000000, -0.000000000000000000 ) ) ;
#126486=EDGE_CURVE ( 'NONE', #35924, #66203, #117482, .T. ) ;
#126487=VERTEX_POINT ( 'NONE', #25618 ) ;
#126488=AXIS2_PLACEMENT_3D ( 'NONE', #7548, #40920, #59913 ) ;
#126489=AXIS2_PLACEMENT_3D ( 'NONE', #43509, #83428, #91298 ) ;
#126490=EDGE_LOOP ( 'NONE', ( #9823, #92778, #99676, #111066 ) ) ;
#126491=PLANE ( 'NONE',  #40157 ) ;
#126492=ORIENTED_EDGE ( 'NONE', *, *, #119633, .T. ) ;
#126493=DIRECTION ( 'NONE',  ( -0.000000000000000000, 1.000000000000000000, -0.000000000000000000 ) ) ;
#126494=CARTESIAN_POINT ( 'NONE',  ( 11.24999999999991118, 12.50000000000000000, 5.802370205355744659 ) ) ;
#126495=EDGE_LOOP ( 'NONE', ( #124688, #40633, #71850, #53133 ) ) ;
#126497=DIRECTION ( 'NONE',  ( 0.000000000000000000, 1.000000000000000000, 0.000000000000000000 ) ) ;
#126498=CARTESIAN_POINT ( 'NONE',  ( -12.09999999999999609, 12.50000000000000000, -5.022947341949751454 ) ) ;
#126499=AXIS2_PLACEMENT_3D ( 'NONE', #113224, #105996, #94235 ) ;
#126500=CARTESIAN_POINT ( 'NONE',  ( 11.64999999999990443, 2.500000000000000000, 2.757883832488649656 ) ) ;
#126501=ORIENTED_EDGE ( 'NONE', *, *, #35514, .T. ) ;
#126502=AXIS2_PLACEMENT_3D ( 'NONE', #122062, #39653, #101773 ) ;
#126503=DIRECTION ( 'NONE',  ( 0.000000000000000000, 1.000000000000000000, 0.000000000000000000 ) ) ;
#126504=DIRECTION ( 'NONE',  ( -0.000000000000000000, -1.000000000000000000, -0.000000000000000000 ) ) ;
#126505=AXIS2_PLACEMENT_3D ( 'NONE', #77523, #19911, #97170 ) ;
#126506=ORIENTED_EDGE ( 'NONE', *, *, #124508, .F. ) ;
#126507=CIRCLE ( 'NONE', #30379, 0.1000000000000002554 ) ;
#126508=CARTESIAN_POINT ( 'NONE',  ( 9.999999999999952038, 12.50000000000000000, -2.276824562219559311E-15 ) ) ;
#126510=CARTESIAN_POINT ( 'NONE',  ( 3.549999999999940314, 12.50000000000000000, 6.776507416713035248 ) ) ;
#126511=CONICAL_SURFACE ( 'NONE', #76337, 0.1000000000000002554, 0.003490658503988666988 ) ;
#126512=CONICAL_SURFACE ( 'NONE', #3185, 0.09999999999999982514, 0.003490658503988666988 ) ;
#126513=ORIENTED_EDGE ( 'NONE', *, *, #106024, .F. ) ;
#126514=CIRCLE ( 'NONE', #70080, 0.1000000000000002554 ) ;
#126515=FACE_OUTER_BOUND ( 'NONE', #99853, .T. ) ;
#126516=AXIS2_PLACEMENT_3D ( 'NONE', #1071, #41027, #10257 ) ;
#126517=ORIENTED_EDGE ( 'NONE', *, *, #116074, .F. ) ;
#126518=PLANE ( 'NONE',  #45872 ) ;
#126519=DIRECTION ( 'NONE',  ( 0.000000000000000000, 0.000000000000000000, -1.000000000000000000 ) ) ;
#126520=PLANE ( 'NONE',  #41284 ) ;
#126521=EDGE_LOOP ( 'NONE', ( #92373, #102304, #58109, #61047 ) ) ;
#126522=AXIS2_PLACEMENT_3D ( 'NONE', #44191, #104411, #74955 ) ;
#126523=CIRCLE ( 'NONE', #11501, 0.06509327318403745899 ) ;
#126524=EDGE_CURVE ( 'NONE', #9000, #35674, #65277, .T. ) ;
#126525=DIRECTION ( 'NONE',  ( 0.000000000000000000, 0.000000000000000000, -1.000000000000000000 ) ) ;
#126526=LINE ( 'NONE', #55839, #51616 ) ;
#126527=AXIS2_PLACEMENT_3D ( 'NONE', #118900, #109053, #19396 ) ;
#126528=EDGE_LOOP ( 'NONE', ( #91272, #5294, #15597, #96421 ) ) ;
#126529=EDGE_CURVE ( 'NONE', #107252, #54196, #45288, .T. ) ;
#126530=ADVANCED_FACE ( 'NONE', ( #44633 ), #114649, .T. ) ;
#126531=EDGE_LOOP ( 'NONE', ( #55677, #103590, #100765, #40934 ) ) ;
#126532=CARTESIAN_POINT ( 'NONE',  ( 11.04999999999990834, 12.50000000000000000, -6.841600689897077814 ) ) ;
#126533=VERTEX_POINT ( 'NONE', #85828 ) ;
#126534=DIRECTION ( 'NONE',  ( 0.000000000000000000, -0.9999939076577903929, 0.003490651415223739937 ) ) ;
#126535=DIRECTION ( 'NONE',  ( -0.000000000000000000, 1.000000000000000000, -0.000000000000000000 ) ) ;
#126536=EDGE_CURVE ( 'NONE', #1046, #22334, #104193, .T. ) ;
#126537=ADVANCED_FACE ( 'NONE', ( #84557 ), #64263, .T. ) ;
#126538=ORIENTED_EDGE ( 'NONE', *, *, #90046, .F. ) ;
#126539=VERTEX_POINT ( 'NONE', #95029 ) ;
#126540=ADVANCED_FACE ( 'NONE', ( #65555 ), #111233, .T. ) ;
#126541=CARTESIAN_POINT ( 'NONE',  ( 3.099999999999945466, 2.500000000000000000, -3.883716857408426648 ) ) ;
#126542=DIRECTION ( 'NONE',  ( -4.274815082592931898E-19, -0.9999939076577903929, -0.003490651415223739937 ) ) ;
#126543=CIRCLE ( 'NONE', #65985, 0.06509327318403745899 ) ;
#126544=ORIENTED_EDGE ( 'NONE', *, *, #126845, .F. ) ;
#126545=DIRECTION ( 'NONE',  ( 0.000000000000000000, 1.000000000000000000, 0.000000000000000000 ) ) ;
#126546=CARTESIAN_POINT ( 'NONE',  ( -3.350000000000028955, 12.50000000000000000, 2.099970236277060032 ) ) ;
#126547=CARTESIAN_POINT ( 'NONE',  ( 3.749999999999978684, 12.50000000000000000, -6.430097255199264339 ) ) ;
#126548=LINE ( 'NONE', #108176, #55072 ) ;
#126549=CARTESIAN_POINT ( 'NONE',  ( -15.19999999999998153, 12.50000000000000000, -0.3464101615137759604 ) ) ;
#126550=CIRCLE ( 'NONE', #1150, 0.06509327318403745899 ) ;
#126551=CARTESIAN_POINT ( 'NONE',  ( 10.84999999999990905, 2.500000000000000000, -6.495190528383302464 ) ) ;
#126552=AXIS2_PLACEMENT_3D ( 'NONE', #101751, #13991, #103691 ) ;
#126553=CIRCLE ( 'NONE', #111982, 0.1000000000000000472 ) ;
#126554=EDGE_LOOP ( 'NONE', ( #100626, #123367 ) ) ;
#126555=ORIENTED_EDGE ( 'NONE', *, *, #64653, .T. ) ;
#126556=ORIENTED_EDGE ( 'NONE', *, *, #49599, .F. ) ;
#126557=ORIENTED_EDGE ( 'NONE', *, *, #20443, .T. ) ;
#126558=CARTESIAN_POINT ( 'NONE',  ( 6.049999999999935874, 2.500000000000000000, -6.841600689897077814 ) ) ;
#126559=DIRECTION ( 'NONE',  ( 0.000000000000000000, 0.000000000000000000, 1.000000000000000000 ) ) ;
#126560=CARTESIAN_POINT ( 'NONE',  ( -1.224646799147353269E-17, 2.500000000000000000, -0.1000000000000000056 ) ) ;
#126561=EDGE_LOOP ( 'NONE', ( #87908, #80624 ) ) ;
#126562=FACE_BOUND ( 'NONE', #10376, .T. ) ;
#126563=DIRECTION ( 'NONE',  ( 0.000000000000000000, 1.000000000000000000, 0.000000000000000000 ) ) ;
#126564=CARTESIAN_POINT ( 'NONE',  ( 10.84999999999991260, 12.50000000000000000, -2.165063509461101710 ) ) ;
#126565=AXIS2_PLACEMENT_3D ( 'NONE', #34767, #103493, #3354 ) ;
#126566=CARTESIAN_POINT ( 'NONE',  ( -1.450000000000036371, 2.500000000000000000, 6.741600689897071952 ) ) ;
#126567=DIRECTION ( 'NONE',  ( 0.000000000000000000, 1.000000000000000000, 0.000000000000000000 ) ) ;
#126568=CONICAL_SURFACE ( 'NONE', #38861, 0.09999999999999982514, 0.003490658503988666988 ) ;
#126569=CARTESIAN_POINT ( 'NONE',  ( 11.64999999999990621, 2.500000000000000000, 6.495190528383297135 ) ) ;
#126570=DIRECTION ( 'NONE',  ( 0.000000000000000000, -0.000000000000000000, 1.000000000000000000 ) ) ;
#126571=CARTESIAN_POINT ( 'NONE',  ( -7.300000000000016698, 12.50000000000000000, -0.3464101615137783474 ) ) ;
#126572=DIRECTION ( 'NONE',  ( 0.000000000000000000, 1.000000000000000000, 0.000000000000000000 ) ) ;
#126573=CARTESIAN_POINT ( 'NONE',  ( 7.299999999999927880, 2.500000000000000000, -4.576537180435977348 ) ) ;
#126574=CARTESIAN_POINT ( 'NONE',  ( 6.249999999999967137, 12.50000000000000000, -2.099970236277064473 ) ) ;
#126575=AXIS2_PLACEMENT_3D ( 'NONE', #14624, #44766, #95149 ) ;
#126576=EDGE_LOOP ( 'NONE', ( #120111, #48691 ) ) ;
#126577=VERTEX_POINT ( 'NONE', #54440 ) ;
#126578=AXIS2_PLACEMENT_3D ( 'NONE', #64414, #76177, #96437 ) ;
#126579=ORIENTED_EDGE ( 'NONE', *, *, #123626, .T. ) ;
#126580=VERTEX_POINT ( 'NONE', #26925 ) ;
#126581=DIRECTION ( 'NONE',  ( 0.000000000000000000, 1.000000000000000000, 0.000000000000000000 ) ) ;
#126582=EDGE_CURVE ( 'NONE', #90407, #51178, #54814, .T. ) ;
#126583=CARTESIAN_POINT ( 'NONE',  ( -10.40000000000000213, 12.50000000000000000, -4.330127018922197202 ) ) ;
#126585=ORIENTED_EDGE ( 'NONE', *, *, #106676, .F. ) ;
#126586=ORIENTED_EDGE ( 'NONE', *, *, #56555, .F. ) ;
#126587=VERTEX_POINT ( 'NONE', #116580 ) ;
#126588=ADVANCED_FACE ( 'NONE', ( #75365 ), #48574, .T. ) ;
#126589=DIRECTION ( 'NONE',  ( -0.000000000000000000, -1.000000000000000000, -0.000000000000000000 ) ) ;
#126590=AXIS2_PLACEMENT_3D ( 'NONE', #9705, #129508, #39828 ) ;
#126591=CARTESIAN_POINT ( 'NONE',  ( 11.75764115780431851, -2.499999999999999112, 7.679135278101805184 ) ) ;
#126592=DIRECTION ( 'NONE',  ( 0.000000000000000000, 0.000000000000000000, -1.000000000000000000 ) ) ;
#126593=DIRECTION ( 'NONE',  ( 0.000000000000000000, -0.9999939076577903929, 0.003490651415223739937 ) ) ;
#126594=ADVANCED_FACE ( 'NONE', ( #36107 ), #86197, .T. ) ;
#126595=DIRECTION ( 'NONE',  ( -4.274815082592931898E-19, -0.9999939076577903929, -0.003490651415223739937 ) ) ;
#126597=AXIS2_PLACEMENT_3D ( 'NONE', #7130, #107279, #37894 ) ;
#126598=ORIENTED_EDGE ( 'NONE', *, *, #114119, .T. ) ;
#126599=ADVANCED_FACE ( 'NONE', ( #126418 ), #63231, .T. ) ;
#126600=EDGE_CURVE ( 'NONE', #71330, #109372, #15076, .T. ) ;
#126601=EDGE_LOOP ( 'NONE', ( #83544, #43773, #78316, #37739 ) ) ;
#126602=EDGE_CURVE ( 'NONE', #118967, #17267, #117202, .T. ) ;
#126603=CIRCLE ( 'NONE', #70163, 0.06509327318403745899 ) ;
#126604=VERTEX_POINT ( 'NONE', #30161 ) ;
#126605=ORIENTED_EDGE ( 'NONE', *, *, #52357, .T. ) ;
#126606=AXIS2_PLACEMENT_3D ( 'NONE', #28442, #119375, #18607 ) ;
#126607=DIRECTION ( 'NONE',  ( -0.000000000000000000, -1.000000000000000000, -0.000000000000000000 ) ) ;
#126608=ORIENTED_EDGE ( 'NONE', *, *, #124508, .T. ) ;
#126609=VERTEX_POINT ( 'NONE', #88401 ) ;
#126610=EDGE_CURVE ( 'NONE', #19230, #117173, #44357, .T. ) ;
#126611=CARTESIAN_POINT ( 'NONE',  ( 11.44999999999990514, 12.50000000000000000, 2.511473670974873507 ) ) ;
#126612=AXIS2_PLACEMENT_3D ( 'NONE', #28907, #6015, #117241 ) ;
#126613=CARTESIAN_POINT ( 'NONE',  ( -8.749999999999975131, 2.500000000000000000, 2.065063509461097624 ) ) ;
#126614=DIRECTION ( 'NONE',  ( -0.000000000000000000, -1.000000000000000000, -0.000000000000000000 ) ) ;
#126615=PLANE ( 'NONE',  #73444 ) ;
#126616=CONICAL_SURFACE ( 'NONE', #17837, 0.1000000000000002554, 0.003490658503988666988 ) ;
#126617=FACE_OUTER_BOUND ( 'NONE', #58580, .T. ) ;
#126618=VERTEX_POINT ( 'NONE', #128371 ) ;
#126619=LINE ( 'NONE', #35654, #103354 ) ;
#126620=CONICAL_SURFACE ( 'NONE', #91196, 0.1000000000000000056, 0.003490658503988666988 ) ;
#126621=CIRCLE ( 'NONE', #72251, 0.09999999999999982514 ) ;
#126622=ORIENTED_EDGE ( 'NONE', *, *, #5831, .F. ) ;
#126623=DIRECTION ( 'NONE',  ( -0.000000000000000000, -1.000000000000000000, -0.000000000000000000 ) ) ;
#126624=CIRCLE ( 'NONE', #70181, 0.1000000000000002554 ) ;
#126625=ORIENTED_EDGE ( 'NONE', *, *, #14245, .F. ) ;
#126627=DIRECTION ( 'NONE',  ( -4.274815082592931898E-19, -0.9999939076577903929, -0.003490651415223739937 ) ) ;
#126628=CIRCLE ( 'NONE', #107742, 0.1000000000000000056 ) ;
#126629=ORIENTED_EDGE ( 'NONE', *, *, #2345, .T. ) ;
#126630=DIRECTION ( 'NONE',  ( 0.000000000000000000, 1.000000000000000000, 0.000000000000000000 ) ) ;
#126631=FACE_OUTER_BOUND ( 'NONE', #102425, .T. ) ;
#126632=ORIENTED_EDGE ( 'NONE', *, *, #55855, .F. ) ;
#126633=CARTESIAN_POINT ( 'NONE',  ( 11.64999999999990443, 12.50000000000000000, 2.857883832488649301 ) ) ;
#126634=ORIENTED_EDGE ( 'NONE', *, *, #78735, .T. ) ;
#126635=ORIENTED_EDGE ( 'NONE', *, *, #98185, .F. ) ;
#126636=FACE_OUTER_BOUND ( 'NONE', #124795, .T. ) ;
#126637=CARTESIAN_POINT ( 'NONE',  ( 8.549999999999924327, 2.500000000000000000, -6.741600689897077281 ) ) ;
#126639=AXIS2_PLACEMENT_3D ( 'NONE', #83108, #122385, #113852 ) ;
#126640=DIRECTION ( 'NONE',  ( 0.000000000000000000, -1.000000000000000000, 0.000000000000000000 ) ) ;
#126641=DIRECTION ( 'NONE',  ( 0.000000000000000000, -0.9999939076577903929, 0.003490651415223739937 ) ) ;
#126642=EDGE_CURVE ( 'NONE', #119412, #57054, #84063, .T. ) ;
#126643=CARTESIAN_POINT ( 'NONE',  ( -11.84999999999999609, 2.500000000000000000, 6.841600689897072485 ) ) ;
#126644=CIRCLE ( 'NONE', #49294, 0.09999999999999982514 ) ;
#126645=CONICAL_SURFACE ( 'NONE', #22198, 0.09999999999999982514, 0.003490658503988666988 ) ;
#126646=VERTEX_POINT ( 'NONE', #20330 ) ;
#126647=CIRCLE ( 'NONE', #91131, 0.06509327318403745899 ) ;
#126648=CARTESIAN_POINT ( 'NONE',  ( 48.83353579394137967, 2.320413785907065485, -5.300554616748716974 ) ) ;
#126649=AXIS2_PLACEMENT_3D ( 'NONE', #77902, #35423, #37988 ) ;
#126650=ORIENTED_EDGE ( 'NONE', *, *, #18743, .F. ) ;
#126651=CARTESIAN_POINT ( 'NONE',  ( -8.950000000000004619, 12.50000000000000000, 6.148780366869520897 ) ) ;
#126652=DIRECTION ( 'NONE',  ( 0.000000000000000000, 0.000000000000000000, -1.000000000000000000 ) ) ;
#126653=CARTESIAN_POINT ( 'NONE',  ( 2.699999999999946443, 2.500000000000000000, 0.3464101615137735735 ) ) ;
#126654=CARTESIAN_POINT ( 'NONE',  ( 8.349999999999919709, 2.500000000000000000, 5.902370205355745192 ) ) ;
#126655=CARTESIAN_POINT ( 'NONE',  ( 10.59999999999991260, 12.50000000000000000, 0.3464101615137735735 ) ) ;
#126656=ORIENTED_EDGE ( 'NONE', *, *, #127682, .T. ) ;
#126657=CIRCLE ( 'NONE', #13764, 0.09999999999999982514 ) ;
#126658=AXIS2_PLACEMENT_3D ( 'NONE', #60287, #683, #68783 ) ;
#126659=CONICAL_SURFACE ( 'NONE', #95356, 0.1000000000000002554, 0.003490658503988666988 ) ;
#126660=CARTESIAN_POINT ( 'NONE',  ( 3.949999999999939782, 2.500000000000000000, 2.511473670974873507 ) ) ;
#126661=DIRECTION ( 'NONE',  ( 0.000000000000000000, 1.000000000000000000, 0.000000000000000000 ) ) ;
#126662=ORIENTED_EDGE ( 'NONE', *, *, #6202, .T. ) ;
#126663=CARTESIAN_POINT ( 'NONE',  ( 3.749999999999942268, 2.500000000000000000, -1.572243186433550211 ) ) ;
#126664=AXIS2_PLACEMENT_3D ( 'NONE', #26257, #85165, #84522 ) ;
#126665=AXIS2_PLACEMENT_3D ( 'NONE', #31589, #102265, #72805 ) ;
#126666=ORIENTED_EDGE ( 'NONE', *, *, #72040, .T. ) ;
#126668=DIRECTION ( 'NONE',  ( 0.000000000000000000, 1.000000000000000000, 0.000000000000000000 ) ) ;
#126669=VERTEX_POINT ( 'NONE', #79887 ) ;
#126670=CARTESIAN_POINT ( 'NONE',  ( 10.59999999999990905, 12.50000000000000000, -4.676537180435978769 ) ) ;
#126671=DIRECTION ( 'NONE',  ( -4.274815082592931898E-19, -0.9999939076577903929, -0.003490651415223739937 ) ) ;
#126672=CARTESIAN_POINT ( 'NONE',  ( 7.899999999999924860, 2.500000000000000000, 3.537306695894645081 ) ) ;
#126673=ORIENTED_EDGE ( 'NONE', *, *, #122241, .T. ) ;
#126674=EDGE_CURVE ( 'NONE', #129385, #94750, #56855, .T. ) ;
#126675=FACE_BOUND ( 'NONE', #121082, .T. ) ;
#126676=CARTESIAN_POINT ( 'NONE',  ( -4.600000000000024514, 2.500000000000000000, 0.7928203230275495672 ) ) ;
#126677=ORIENTED_EDGE ( 'NONE', *, *, #55869, .T. ) ;
#126678=DIRECTION ( 'NONE',  ( -0.000000000000000000, 1.000000000000000000, -0.000000000000000000 ) ) ;
#126679=EDGE_CURVE ( 'NONE', #107267, #33453, #57681, .T. ) ;
#126680=DIRECTION ( 'NONE',  ( 0.000000000000000000, -0.000000000000000000, 1.000000000000000000 ) ) ;
#126681=EDGE_CURVE ( 'NONE', #12101, #62381, #423, .T. ) ;
#126682=ORIENTED_EDGE ( 'NONE', *, *, #91505, .T. ) ;
#126683=AXIS2_PLACEMENT_3D ( 'NONE', #3417, #36109, #76023 ) ;
#126684=EDGE_LOOP ( 'NONE', ( #9208, #33290, #92446, #38038 ) ) ;
#126685=CIRCLE ( 'NONE', #66037, 0.06509327318403745899 ) ;
#126686=ORIENTED_EDGE ( 'NONE', *, *, #58168, .F. ) ;
#126687=DIRECTION ( 'NONE',  ( -0.000000000000000000, 1.000000000000000000, -0.000000000000000000 ) ) ;
#126688=FACE_OUTER_BOUND ( 'NONE', #12827, .T. ) ;
#126689=EDGE_CURVE ( 'NONE', #27988, #93997, #4613, .T. ) ;
#126690=EDGE_CURVE ( 'NONE', #44951, #14578, #110000, .T. ) ;
#126691=DIRECTION ( 'NONE',  ( 0.000000000000000000, 1.000000000000000000, 0.000000000000000000 ) ) ;
#126692=EDGE_CURVE ( 'NONE', #4337, #74953, #59135, .T. ) ;
#126693=FACE_BOUND ( 'NONE', #110848, .T. ) ;
#126694=EDGE_LOOP ( 'NONE', ( #64948, #99859, #72643, #99439 ) ) ;
#126695=ADVANCED_FACE ( 'NONE', ( #89072 ), #9215, .T. ) ;
#126696=EDGE_CURVE ( 'NONE', #5490, #13290, #60278, .T. ) ;
#126697=CARTESIAN_POINT ( 'NONE',  ( -9.800000000000006040, 2.500000000000000000, 0.2464101615137735679 ) ) ;
#126698=FACE_OUTER_BOUND ( 'NONE', #27355, .T. ) ;
#126699=CIRCLE ( 'NONE', #109974, 0.09999999999999982514 ) ;
#126700=DIRECTION ( 'NONE',  ( 0.000000000000000000, 1.000000000000000000, 0.000000000000000000 ) ) ;
#126701=FACE_OUTER_BOUND ( 'NONE', #23329, .T. ) ;
#126702=DIRECTION ( 'NONE',  ( -0.000000000000000000, -1.000000000000000000, -0.000000000000000000 ) ) ;
#126704=DIRECTION ( 'NONE',  ( 0.000000000000000000, 0.000000000000000000, 1.000000000000000000 ) ) ;
#126705=CARTESIAN_POINT ( 'NONE',  ( -2.900000000000030553, 2.500000000000000000, 5.022947341949748790 ) ) ;
#126706=AXIS2_PLACEMENT_3D ( 'NONE', #86543, #7330, #126482 ) ;
#126707=EDGE_CURVE ( 'NONE', #47870, #101225, #100179, .T. ) ;
#126708=AXIS2_PLACEMENT_3D ( 'NONE', #87138, #117223, #77968 ) ;
#126709=VERTEX_POINT ( 'NONE', #79260 ) ;
#126710=ORIENTED_EDGE ( 'NONE', *, *, #94932, .F. ) ;
#126711=EDGE_LOOP ( 'NONE', ( #41002, #3870, #116143, #129433 ) ) ;
#126712=VERTEX_POINT ( 'NONE', #59635 ) ;
#126713=EDGE_LOOP ( 'NONE', ( #111052, #13607, #54833, #43816 ) ) ;
#126714=CARTESIAN_POINT ( 'NONE',  ( -10.84999999999999964, 2.500000000000000000, 2.957883832488649389 ) ) ;
#126715=CARTESIAN_POINT ( 'NONE',  ( 0.6499999999999561684, 2.500000000000000000, -2.611473670974877592 ) ) ;
#126716=VERTEX_POINT ( 'NONE', #108056 ) ;
#126717=FACE_BOUND ( 'NONE', #13407, .T. ) ;
#126718=CARTESIAN_POINT ( 'NONE',  ( 5.849999999999934808, 12.50000000000000000, -5.867463478539787225 ) ) ;
#126719=CARTESIAN_POINT ( 'NONE',  ( -13.09999999999999254, 2.500000000000000000, -0.2464101615137741230 ) ) ;
#126720=DIRECTION ( 'NONE',  ( 0.000000000000000000, 0.000000000000000000, 1.000000000000000000 ) ) ;
#126721=CARTESIAN_POINT ( 'NONE',  ( -1.650000000000034772, 12.50000000000000000, 1.472243186433545459 ) ) ;
#126722=CARTESIAN_POINT ( 'NONE',  ( -0.8500000000000386136, 12.50000000000000000, 2.857883832488649301 ) ) ;
#126723=AXIS2_PLACEMENT_3D ( 'NONE', #12253, #53494, #23359 ) ;
#126725=CARTESIAN_POINT ( 'NONE',  ( 17.46224679592722495, -2.499999999999374278, 5.244174652594745467 ) ) ;
#126726=ORIENTED_EDGE ( 'NONE', *, *, #92085, .F. ) ;
#126728=VECTOR ( 'NONE', #86018, 1000.000000000000000 ) ;
#126729=VERTEX_POINT ( 'NONE', #99543 ) ;
#126730=ORIENTED_EDGE ( 'NONE', *, *, #89155, .F. ) ;
#126731=FACE_OUTER_BOUND ( 'NONE', #40610, .T. ) ;
#126732=DIRECTION ( 'NONE',  ( 0.000000000000000000, 0.000000000000000000, 1.000000000000000000 ) ) ;
#126733=CARTESIAN_POINT ( 'NONE',  ( 8.749999999999923617, 12.50000000000000000, -7.122917578226816815 ) ) ;
#126734=EDGE_CURVE ( 'NONE', #11709, #113, #65364, .T. ) ;
#126735=EDGE_LOOP ( 'NONE', ( #1681, #111403 ) ) ;
#126736=CARTESIAN_POINT ( 'NONE',  ( 13.92826132181788346, 2.499999999999999556, -6.790916467785696575 ) ) ;
#126737=VECTOR ( 'NONE', #72139, 1000.000000000000000 ) ;
#126738=EDGE_CURVE ( 'NONE', #71628, #127250, #123861, .T. ) ;
#126739=AXIS2_PLACEMENT_3D ( 'NONE', #112708, #11914, #119948 ) ;
#126740=DIRECTION ( 'NONE',  ( -0.000000000000000000, 1.000000000000000000, -0.000000000000000000 ) ) ;
#126741=CIRCLE ( 'NONE', #76649, 0.06509327318403745899 ) ;
#126742=ADVANCED_FACE ( 'NONE', ( #58335 ), #70074, .T. ) ;
#126743=DIRECTION ( 'NONE',  ( 0.000000000000000000, -0.9999939076577903929, 0.003490651415223739937 ) ) ;
#126745=CARTESIAN_POINT ( 'NONE',  ( 12.29999999999990479, 12.50000000000000000, 4.741630453620009789 ) ) ;
#126746=DIRECTION ( 'NONE',  ( 0.000000000000000000, 0.000000000000000000, 1.000000000000000000 ) ) ;
#126747=DIRECTION ( 'NONE',  ( -4.274815082592931898E-19, -0.9999939076577903929, -0.003490651415223739937 ) ) ;
#126748=EDGE_CURVE ( 'NONE', #102161, #26161, #107135, .T. ) ;
#126749=VERTEX_POINT ( 'NONE', #102732 ) ;
#126750=CARTESIAN_POINT ( 'NONE',  ( 11.64999999999990443, 2.500000000000000000, 1.472243186433545459 ) ) ;
#126751=CIRCLE ( 'NONE', #118328, 0.1000000000000002554 ) ;
#126753=VERTEX_POINT ( 'NONE', #40639 ) ;
#126754=AXIS2_PLACEMENT_3D ( 'NONE', #93432, #94075, #111106 ) ;
#126755=CIRCLE ( 'NONE', #43150, 0.06509327318403745899 ) ;
#126756=EDGE_CURVE ( 'NONE', #31984, #11223, #111253, .T. ) ;
#126757=ORIENTED_EDGE ( 'NONE', *, *, #48388, .F. ) ;
#126758=DIRECTION ( 'NONE',  ( 0.000000000000000000, -0.000000000000000000, 1.000000000000000000 ) ) ;
#126759=CARTESIAN_POINT ( 'NONE',  ( 0.3999999999999619971, 2.500000000000000000, 0.09999999999999989453 ) ) ;
#126760=DIRECTION ( 'NONE',  ( 0.000000000000000000, 1.000000000000000000, 0.000000000000000000 ) ) ;
#126761=ORIENTED_EDGE ( 'NONE', *, *, #73616, .F. ) ;
#126762=ADVANCED_FACE ( 'NONE', ( #92943 ), #122402, .T. ) ;
#126763=ORIENTED_EDGE ( 'NONE', *, *, #104379, .T. ) ;
#126764=DIRECTION ( 'NONE',  ( 0.000000000000000000, 1.000000000000000000, 0.000000000000000000 ) ) ;
#126765=CARTESIAN_POINT ( 'NONE',  ( -1.650000000000034772, 2.500000000000000000, 6.595190528383296780 ) ) ;
#126766=CARTESIAN_POINT ( 'NONE',  ( -5.000000000000022204, 12.50000000000000000, 3.572213422710607489 ) ) ;
#126767=ORIENTED_EDGE ( 'NONE', *, *, #90846, .T. ) ;
#126768=ORIENTED_EDGE ( 'NONE', *, *, #114447, .F. ) ;
#126769=DIRECTION ( 'NONE',  ( 0.000000000000000000, 1.000000000000000000, 0.000000000000000000 ) ) ;
#126770=ORIENTED_EDGE ( 'NONE', *, *, #40718, .T. ) ;
#126771=DIRECTION ( 'NONE',  ( -4.274815082592931898E-19, -0.9999939076577903929, -0.003490651415223739937 ) ) ;
#126772=DIRECTION ( 'NONE',  ( -0.000000000000000000, -1.000000000000000000, -0.000000000000000000 ) ) ;
#126773=ORIENTED_EDGE ( 'NONE', *, *, #35361, .F. ) ;
#126774=PLANE ( 'NONE',  #6369 ) ;
#126775=CARTESIAN_POINT ( 'NONE',  ( -5.850000000000018296, 12.50000000000000000, 2.857883832488649301 ) ) ;
#126776=DIRECTION ( 'NONE',  ( 0.000000000000000000, 0.000000000000000000, 1.000000000000000000 ) ) ;
#126777=EDGE_CURVE ( 'NONE', #74876, #10395, #22911, .T. ) ;
#126778=DIRECTION ( 'NONE',  ( 0.000000000000000000, -0.000000000000000000, 1.000000000000000000 ) ) ;
#126779=VERTEX_POINT ( 'NONE', #3265 ) ;
#126780=DIRECTION ( 'NONE',  ( 0.000000000000000000, -0.000000000000000000, 1.000000000000000000 ) ) ;
#126782=CIRCLE ( 'NONE', #39068, 0.06509327318403745899 ) ;
#126783=DIRECTION ( 'NONE',  ( -0.000000000000000000, -1.000000000000000000, -0.000000000000000000 ) ) ;
#126784=ORIENTED_EDGE ( 'NONE', *, *, #64636, .T. ) ;
#126785=ORIENTED_EDGE ( 'NONE', *, *, #58208, .F. ) ;
#126787=DIRECTION ( 'NONE',  ( 0.000000000000000000, 0.000000000000000000, -1.000000000000000000 ) ) ;
#126788=LINE ( 'NONE', #46279, #74030 ) ;
#126789=CARTESIAN_POINT ( 'NONE',  ( 4.199999999999941558, 2.500000000000000000, -4.330127018922201643 ) ) ;
#126790=CARTESIAN_POINT ( 'NONE',  ( 2.499999999999981792, 2.500000000000000000, 4.430127018922196847 ) ) ;
#126791=AXIS2_PLACEMENT_3D ( 'NONE', #74652, #74018, #34097 ) ;
#126792=CARTESIAN_POINT ( 'NONE',  ( -1.050000000000037792, 12.50000000000000000, 6.148780366869520009 ) ) ;
#126793=AXIS2_PLACEMENT_3D ( 'NONE', #76316, #26571, #35745 ) ;
#126794=FACE_OUTER_BOUND ( 'NONE', #56508, .T. ) ;
#126796=DIRECTION ( 'NONE',  ( 0.000000000000000000, 1.000000000000000000, 0.000000000000000000 ) ) ;
#126797=DIRECTION ( 'NONE',  ( -0.000000000000000000, -1.000000000000000000, -0.000000000000000000 ) ) ;
#126798=DIRECTION ( 'NONE',  ( 0.000000000000000000, 1.000000000000000000, 0.000000000000000000 ) ) ;
#126799=AXIS2_PLACEMENT_3D ( 'NONE', #82541, #122466, #32804 ) ;
#126800=CONICAL_SURFACE ( 'NONE', #13910, 0.1000000000000002554, 0.003490658503988666988 ) ;
#126801=CIRCLE ( 'NONE', #124657, 0.1000000000000002554 ) ;
#126802=ORIENTED_EDGE ( 'NONE', *, *, #73218, .F. ) ;
#126803=DIRECTION ( 'NONE',  ( 0.000000000000000000, 0.000000000000000000, 1.000000000000000000 ) ) ;
#126804=ADVANCED_FACE ( 'NONE', ( #81809 ), #25667, .T. ) ;
#126805=DIRECTION ( 'NONE',  ( 0.000000000000000000, 1.000000000000000000, 0.000000000000000000 ) ) ;
#126806=CARTESIAN_POINT ( 'NONE',  ( 9.349999999999916156, 12.50000000000000000, 6.906693963081109722 ) ) ;
#126807=DIRECTION ( 'NONE',  ( -0.000000000000000000, 1.000000000000000000, -0.000000000000000000 ) ) ;
#126808=ORIENTED_EDGE ( 'NONE', *, *, #84249, .F. ) ;
#126809=DIRECTION ( 'NONE',  ( -0.000000000000000000, 1.000000000000000000, -0.000000000000000000 ) ) ;
#126811=DIRECTION ( 'NONE',  ( 0.000000000000000000, -0.9999939076577903929, 0.003490651415223739937 ) ) ;
#126812=EDGE_LOOP ( 'NONE', ( #91851, #11002 ) ) ;
#126813=AXIS2_PLACEMENT_3D ( 'NONE', #22115, #62023, #52195 ) ;
#126814=ORIENTED_EDGE ( 'NONE', *, *, #91458, .F. ) ;
#126815=AXIS2_PLACEMENT_3D ( 'NONE', #36269, #115426, #125904 ) ;
#126816=CIRCLE ( 'NONE', #30696, 0.06509327318403745899 ) ;
#126817=ORIENTED_EDGE ( 'NONE', *, *, #85616, .T. ) ;
#126818=ORIENTED_EDGE ( 'NONE', *, *, #109843, .T. ) ;
#126819=ORIENTED_EDGE ( 'NONE', *, *, #5073, .F. ) ;
#126820=DIRECTION ( 'NONE',  ( 0.000000000000000000, -0.000000000000000000, 1.000000000000000000 ) ) ;
#126821=VECTOR ( 'NONE', #75663, 1000.000000000000000 ) ;
#126822=CARTESIAN_POINT ( 'NONE',  ( -17.50000000000000000, 1.500000000000000000, 1.734723475976807094E-15 ) ) ;
#126823=CARTESIAN_POINT ( 'NONE',  ( 2.499999999999948930, 12.50000000000000000, -5.022947341949754119 ) ) ;
#126824=CIRCLE ( 'NONE', #28631, 0.1000000000000002554 ) ;
#126825=CARTESIAN_POINT ( 'NONE',  ( 0.7999999999999553024, 2.500000000000000000, -4.430127018922202176 ) ) ;
#126826=VERTEX_POINT ( 'NONE', #43206 ) ;
#126827=CIRCLE ( 'NONE', #93476, 0.09999999999999999167 ) ;
#126828=ADVANCED_FACE ( 'NONE', ( #30812 ), #80054, .T. ) ;
#126829=CARTESIAN_POINT ( 'NONE',  ( 10.39999999999990976, 2.500000000000000000, 4.230127018922196669 ) ) ;
#126830=ORIENTED_EDGE ( 'NONE', *, *, #83718, .T. ) ;
#126831=DIRECTION ( 'NONE',  ( -4.274815082592931898E-19, -0.9999939076577903929, -0.003490651415223739937 ) ) ;
#126832=CARTESIAN_POINT ( 'NONE',  ( -6.050000000000022027, 2.500000000000000000, -6.148780366869526226 ) ) ;
#126833=FACE_OUTER_BOUND ( 'NONE', #120818, .T. ) ;
#126834=CARTESIAN_POINT ( 'NONE',  ( 10.84999999999991260, 12.50000000000000000, -1.472243186433550122 ) ) ;
#126835=AXIS2_PLACEMENT_3D ( 'NONE', #53655, #43213, #20972 ) ;
#126836=EDGE_CURVE ( 'NONE', #125502, #16131, #17232, .T. ) ;
#126837=VERTEX_POINT ( 'NONE', #31445 ) ;
#126838=AXIS2_PLACEMENT_3D ( 'NONE', #88085, #100509, #127404 ) ;
#126839=AXIS2_PLACEMENT_3D ( 'NONE', #3890, #53006, #90987 ) ;
#126840=ORIENTED_EDGE ( 'NONE', *, *, #12761, .F. ) ;
#126841=ORIENTED_EDGE ( 'NONE', *, *, #79165, .T. ) ;
#126842=ORIENTED_EDGE ( 'NONE', *, *, #18256, .F. ) ;
#126843=CARTESIAN_POINT ( 'NONE',  ( 9.199999999999915801, 2.500000000000000000, 4.430127018922196847 ) ) ;
#126844=CARTESIAN_POINT ( 'NONE',  ( 6.249999999999967137, 2.500000000000000000, 6.395190528383296602 ) ) ;
#126845=EDGE_CURVE ( 'NONE', #119064, #104360, #22279, .T. ) ;
#126846=EDGE_CURVE ( 'NONE', #80874, #91490, #100873, .T. ) ;
#126847=LINE ( 'NONE', #86251, #115075 ) ;
#126848=ADVANCED_FACE ( 'NONE', ( #33387 ), #11130, .T. ) ;
#126849=FACE_BOUND ( 'NONE', #124282, .T. ) ;
#126850=EDGE_CURVE ( 'NONE', #33917, #31361, #40362, .T. ) ;
#126851=CARTESIAN_POINT ( 'NONE',  ( 12.49999999999990052, 12.50000000000000000, 0.6277270498435120194 ) ) ;
#126852=DIRECTION ( 'NONE',  ( 0.000000000000000000, 1.000000000000000000, 0.000000000000000000 ) ) ;
#126853=DIRECTION ( 'NONE',  ( 0.000000000000000000, 0.000000000000000000, -1.000000000000000000 ) ) ;
#126854=CARTESIAN_POINT ( 'NONE',  ( -10.65000000000000391, 12.50000000000000000, -6.841600689897075149 ) ) ;
#126855=EDGE_CURVE ( 'NONE', #61868, #1183, #42409, .T. ) ;
#126856=ADVANCED_FACE ( 'NONE', ( #72015 ), #21617, .T. ) ;
#126858=CARTESIAN_POINT ( 'NONE',  ( -8.350000000000008527, 2.500000000000000000, 5.802370205355744659 ) ) ;
#126859=AXIS2_PLACEMENT_3D ( 'NONE', #10950, #90830, #50921 ) ;
#126860=ADVANCED_FACE ( 'NONE', ( #121735 ), #2664, .T. ) ;
#126861=CARTESIAN_POINT ( 'NONE',  ( -0.8500000000000395017, 12.50000000000000000, 6.495190528383297135 ) ) ;
#126862=EDGE_CURVE ( 'NONE', #111547, #126431, #75831, .T. ) ;
#126864=CARTESIAN_POINT ( 'NONE',  ( -11.05000000000000071, 2.500000000000000000, 6.841600689897072485 ) ) ;
#126865=VERTEX_POINT ( 'NONE', #26130 ) ;
#126866=ORIENTED_EDGE ( 'NONE', *, *, #80522, .F. ) ;
#126867=ORIENTED_EDGE ( 'NONE', *, *, #49447, .F. ) ;
#126868=ORIENTED_EDGE ( 'NONE', *, *, #122813, .F. ) ;
#126870=FACE_BOUND ( 'NONE', #36863, .T. ) ;
#126871=ADVANCED_FACE ( 'NONE', ( #113865 ), #54292, .T. ) ;
#126872=DIRECTION ( 'NONE',  ( -0.000000000000000000, 1.000000000000000000, -0.000000000000000000 ) ) ;
#126873=DIRECTION ( 'NONE',  ( -0.000000000000000000, 1.000000000000000000, -0.000000000000000000 ) ) ;
#126874=VECTOR ( 'NONE', #12901, 1000.000000000000000 ) ;
#126875=AXIS2_PLACEMENT_3D ( 'NONE', #126655, #63383, #103311 ) ;
#126876=EDGE_LOOP ( 'NONE', ( #70216, #102831 ) ) ;
#126877=DIRECTION ( 'NONE',  ( 0.000000000000000000, 0.000000000000000000, 1.000000000000000000 ) ) ;
#126878=FACE_OUTER_BOUND ( 'NONE', #9816, .T. ) ;
#126879=ORIENTED_EDGE ( 'NONE', *, *, #126901, .T. ) ;
#126881=DIRECTION ( 'NONE',  ( -4.274815082592931898E-19, -0.9999939076577903929, -0.003490651415223739937 ) ) ;
#126882=AXIS2_PLACEMENT_3D ( 'NONE', #36023, #75935, #115867 ) ;
#126883=AXIS2_PLACEMENT_3D ( 'NONE', #33294, #112486, #1231 ) ;
#126884=ORIENTED_EDGE ( 'NONE', *, *, #86370, .F. ) ;
#126885=DIRECTION ( 'NONE',  ( 0.000000000000000000, 0.000000000000000000, -1.000000000000000000 ) ) ;
#126886=DIRECTION ( 'NONE',  ( 0.000000000000000000, 0.000000000000000000, 1.000000000000000000 ) ) ;
#126887=AXIS2_PLACEMENT_3D ( 'NONE', #60652, #122153, #50821 ) ;
#126888=AXIS2_PLACEMENT_3D ( 'NONE', #115218, #104146, #14454 ) ;
#126889=VERTEX_POINT ( 'NONE', #6441 ) ;
#126890=AXIS2_PLACEMENT_3D ( 'NONE', #92583, #42199, #112227 ) ;
#126891=DIRECTION ( 'NONE',  ( 0.000000000000000000, 0.000000000000000000, 1.000000000000000000 ) ) ;
#126892=DIRECTION ( 'NONE',  ( 0.000000000000000000, 0.000000000000000000, -1.000000000000000000 ) ) ;
#126893=ORIENTED_EDGE ( 'NONE', *, *, #121981, .T. ) ;
#126894=FACE_OUTER_BOUND ( 'NONE', #84969, .T. ) ;
#126895=VERTEX_POINT ( 'NONE', #64750 ) ;
#126896=EDGE_LOOP ( 'NONE', ( #124492, #66880 ) ) ;
#126897=DIRECTION ( 'NONE',  ( 0.000000000000000000, 0.000000000000000000, 1.000000000000000000 ) ) ;
#126898=ORIENTED_EDGE ( 'NONE', *, *, #100947, .T. ) ;
#126899=DIRECTION ( 'NONE',  ( -0.000000000000000000, -1.000000000000000000, -0.000000000000000000 ) ) ;
#126900=DIRECTION ( 'NONE',  ( 0.000000000000000000, 0.000000000000000000, 1.000000000000000000 ) ) ;
#126901=EDGE_CURVE ( 'NONE', #120397, #63967, #64108, .T. ) ;
#126902=EDGE_LOOP ( 'NONE', ( #47372, #95911 ) ) ;
#126903=DIRECTION ( 'NONE',  ( 0.000000000000000000, 0.000000000000000000, -1.000000000000000000 ) ) ;
#126904=EDGE_CURVE ( 'NONE', #2089, #129059, #23613, .T. ) ;
#126905=ORIENTED_EDGE ( 'NONE', *, *, #105334, .T. ) ;
#126906=DIRECTION ( 'NONE',  ( -0.000000000000000000, -1.000000000000000000, -0.000000000000000000 ) ) ;
#126907=CARTESIAN_POINT ( 'NONE',  ( 11.44999999999991047, 2.500000000000000000, -2.511473670974877948 ) ) ;
#126908=DIRECTION ( 'NONE',  ( 0.000000000000000000, 0.000000000000000000, -1.000000000000000000 ) ) ;
#126909=CARTESIAN_POINT ( 'NONE',  ( -6.850000000000017408, 2.500000000000000000, -6.148780366869526226 ) ) ;
#126910=CARTESIAN_POINT ( 'NONE',  ( 17.49101023696816881, 2.144674160806442575, -4.220798295113491250 ) ) ;
#126911=CIRCLE ( 'NONE', #91389, 0.06509327318403741736 ) ;
#126912=CONICAL_SURFACE ( 'NONE', #7763, 0.1000000000000002554, 0.003490658503988666988 ) ;
#126913=ADVANCED_FACE ( 'NONE', ( #5176 ), #29881, .T. ) ;
#126914=ORIENTED_EDGE ( 'NONE', *, *, #34431, .F. ) ;
#126915=VERTEX_POINT ( 'NONE', #126258 ) ;
#126916=CARTESIAN_POINT ( 'NONE',  ( -0.6500000000000394351, 2.500000000000000000, 6.941600689897073018 ) ) ;
#126917=AXIS2_PLACEMENT_3D ( 'NONE', #85297, #26401, #125235 ) ;
#126918=CARTESIAN_POINT ( 'NONE',  ( -7.499999999999980460, 12.50000000000000000, -4.265033745738164406 ) ) ;
#126919=LINE ( 'NONE', #16914, #24963 ) ;
#126920=VERTEX_POINT ( 'NONE', #36611 ) ;
#126921=EDGE_LOOP ( 'NONE', ( #71223, #116146, #128643, #81197 ) ) ;
#126922=VERTEX_POINT ( 'NONE', #85679 ) ;
#126923=CARTESIAN_POINT ( 'NONE',  ( -9.800000000000006040, 2.500000000000000000, -4.576537180435973795 ) ) ;
#126924=CIRCLE ( 'NONE', #129093, 0.06509327318403745899 ) ;
#126925=AXIS2_PLACEMENT_3D ( 'NONE', #43666, #124133, #12237 ) ;
#126926=PLANE ( 'NONE',  #98767 ) ;
#126927=CARTESIAN_POINT ( 'NONE',  ( 9.149999999999916866, 12.50000000000000000, 5.867463478539781896 ) ) ;
#126928=AXIS2_PLACEMENT_3D ( 'NONE', #26846, #87689, #66757 ) ;
#126930=FACE_OUTER_BOUND ( 'NONE', #50272, .T. ) ;
#126932=DIRECTION ( 'NONE',  ( -4.274815082592931898E-19, -0.9999939076577903929, -0.003490651415223739937 ) ) ;
#126933=CARTESIAN_POINT ( 'NONE',  ( 12.69999999999990159, 12.50000000000000000, 4.676537180435972552 ) ) ;
#126934=DIRECTION ( 'NONE',  ( -0.000000000000000000, -1.000000000000000000, -0.000000000000000000 ) ) ;
#126935=CIRCLE ( 'NONE', #35010, 0.09999999999999999167 ) ;
#126936=DIRECTION ( 'NONE',  ( 0.000000000000000000, 0.000000000000000000, 1.000000000000000000 ) ) ;
#126937=ORIENTED_EDGE ( 'NONE', *, *, #39596, .F. ) ;
#126938=CONICAL_SURFACE ( 'NONE', #91417, 0.1000000000000002554, 0.003490658503988666988 ) ;
#126939=CIRCLE ( 'NONE', #47518, 0.09999999999999999167 ) ;
#126940=PLANE ( 'NONE',  #48665 ) ;
#126941=ORIENTED_EDGE ( 'NONE', *, *, #34862, .T. ) ;
#126942=ORIENTED_EDGE ( 'NONE', *, *, #51958, .T. ) ;
#126943=DIRECTION ( 'NONE',  ( 0.000000000000000000, 0.000000000000000000, -1.000000000000000000 ) ) ;
#126944=DIRECTION ( 'NONE',  ( -0.000000000000000000, 1.000000000000000000, -0.000000000000000000 ) ) ;
#126945=LINE ( 'NONE', #47103, #125951 ) ;
#126946=DIRECTION ( 'NONE',  ( -0.000000000000000000, -1.000000000000000000, -0.000000000000000000 ) ) ;
#126947=DIRECTION ( 'NONE',  ( 0.000000000000000000, 0.000000000000000000, 1.000000000000000000 ) ) ;
#126948=FACE_OUTER_BOUND ( 'NONE', #125338, .T. ) ;
#126949=CARTESIAN_POINT ( 'NONE',  ( 3.349999999999941913, 2.500000000000000000, 5.902370205355745192 ) ) ;
#126950=ORIENTED_EDGE ( 'NONE', *, *, #121927, .T. ) ;
#126951=DIRECTION ( 'NONE',  ( 0.000000000000000000, 0.000000000000000000, 1.000000000000000000 ) ) ;
#126952=VECTOR ( 'NONE', #36589, 1000.000000000000000 ) ;
#126953=DIRECTION ( 'NONE',  ( 0.000000000000000000, 1.000000000000000000, 0.000000000000000000 ) ) ;
#126954=ORIENTED_EDGE ( 'NONE', *, *, #129080, .T. ) ;
#126955=ORIENTED_EDGE ( 'NONE', *, *, #47381, .T. ) ;
#126956=EDGE_CURVE ( 'NONE', #30920, #9494, #3897, .T. ) ;
#126957=ORIENTED_EDGE ( 'NONE', *, *, #25363, .F. ) ;
#126958=ADVANCED_FACE ( 'NONE', ( #96145 ), #46392, .T. ) ;
#126959=ORIENTED_EDGE ( 'NONE', *, *, #81010, .T. ) ;
#126960=CARTESIAN_POINT ( 'NONE',  ( -8.150000000000012790, 2.500000000000000000, 2.411473670974873862 ) ) ;
#126961=DIRECTION ( 'NONE',  ( 0.000000000000000000, 0.000000000000000000, 1.000000000000000000 ) ) ;
#126962=EDGE_LOOP ( 'NONE', ( #56459, #100495, #51469, #50528 ) ) ;
#126963=CONICAL_SURFACE ( 'NONE', #1558, 0.09999999999999982514, 0.003490658503988666988 ) ;
#126964=CARTESIAN_POINT ( 'NONE',  ( -0.4000000000000331624, 2.500000000000000000, -0.6928203230275519209 ) ) ;
#126965=AXIS2_PLACEMENT_3D ( 'NONE', #113450, #43445, #4123 ) ;
#126966=CARTESIAN_POINT ( 'NONE',  ( 2.899999999999944844, 2.500000000000000000, 3.637306695894644726 ) ) ;
#126967=DIRECTION ( 'NONE',  ( 0.000000000000000000, 0.000000000000000000, 1.000000000000000000 ) ) ;
#126968=EDGE_LOOP ( 'NONE', ( #56623, #76873, #119238, #106157 ) ) ;
#126969=EDGE_CURVE ( 'NONE', #98359, #20666, #119752, .T. ) ;
#126970=DIRECTION ( 'NONE',  ( 0.000000000000000000, 1.000000000000000000, 0.000000000000000000 ) ) ;
#126971=VECTOR ( 'NONE', #85608, 1000.000000000000000 ) ;
#126972=AXIS2_PLACEMENT_3D ( 'NONE', #83668, #81098, #33916 ) ;
#126973=CARTESIAN_POINT ( 'NONE',  ( 3.549999999999942091, 12.50000000000000000, 2.511473670974873507 ) ) ;
#126974=ORIENTED_EDGE ( 'NONE', *, *, #25323, .F. ) ;
#126975=AXIS2_PLACEMENT_3D ( 'NONE', #9883, #77330, #97613 ) ;
#126976=ORIENTED_EDGE ( 'NONE', *, *, #103206, .T. ) ;
#126977=EDGE_LOOP ( 'NONE', ( #9199, #30705, #94059, #7428 ) ) ;
#126978=FACE_OUTER_BOUND ( 'NONE', #109852, .T. ) ;
#126979=AXIS2_PLACEMENT_3D ( 'NONE', #95260, #63210, #14728 ) ;
#126980=CONICAL_SURFACE ( 'NONE', #70535, 0.1000000000000000472, 0.003490658503988666988 ) ;
#126981=CARTESIAN_POINT ( 'NONE',  ( 2.099999999999947686, 12.50000000000000000, 5.022947341949748790 ) ) ;
#126982=VECTOR ( 'NONE', #4653, 1000.000000000000000 ) ;
#126983=EDGE_CURVE ( 'NONE', #127177, #65511, #10979, .T. ) ;
#126984=ORIENTED_EDGE ( 'NONE', *, *, #66515, .T. ) ;
#126985=DIRECTION ( 'NONE',  ( 0.000000000000000000, 0.000000000000000000, 1.000000000000000000 ) ) ;
#126986=CARTESIAN_POINT ( 'NONE',  ( 1.899999999999951283, 2.500000000000000000, -3.883716857408426648 ) ) ;
#126987=FACE_OUTER_BOUND ( 'NONE', #5201, .T. ) ;
#126988=CARTESIAN_POINT ( 'NONE',  ( 7.699999999999922018, 12.50000000000000000, 0.3464101615137735735 ) ) ;
#126989=EDGE_CURVE ( 'NONE', #124287, #7788, #123656, .T. ) ;
#126990=ORIENTED_EDGE ( 'NONE', *, *, #81181, .F. ) ;
#126991=CONICAL_SURFACE ( 'NONE', #87265, 0.09999999999999999167, 0.003490658503988666988 ) ;
#126992=CARTESIAN_POINT ( 'NONE',  ( -8.750000000000010658, 12.50000000000000000, -7.122917578226811486 ) ) ;
#126993=CONICAL_SURFACE ( 'NONE', #14105, 0.1000000000000000472, 0.003490658503988666988 ) ;
#126994=EDGE_LOOP ( 'NONE', ( #95376, #52144 ) ) ;
#126995=ORIENTED_EDGE ( 'NONE', *, *, #110564, .T. ) ;
#126996=ADVANCED_FACE ( 'NONE', ( #4513 ), #21467, .T. ) ;
#126997=VERTEX_POINT ( 'NONE', #24835 ) ;
#126998=ADVANCED_FACE ( 'NONE', ( #94863 ), #54905, .T. ) ;
#126999=FACE_OUTER_BOUND ( 'NONE', #80788, .T. ) ;
#127000=EDGE_CURVE ( 'NONE', #97467, #104697, #71639, .T. ) ;
#127001=FACE_BOUND ( 'NONE', #96141, .T. ) ;
#127002=CIRCLE ( 'NONE', #87274, 0.06509327318403745899 ) ;
#127003=EDGE_CURVE ( 'NONE', #48809, #89954, #84241, .T. ) ;
#127004=DIRECTION ( 'NONE',  ( 0.000000000000000000, 1.000000000000000000, 0.000000000000000000 ) ) ;
#127005=FACE_OUTER_BOUND ( 'NONE', #85659, .T. ) ;
#127006=VECTOR ( 'NONE', #67904, 1000.000000000000000 ) ;
#127007=PLANE ( 'NONE',  #85705 ) ;
#127008=AXIS2_PLACEMENT_3D ( 'NONE', #82056, #1562, #70958 ) ;
#127009=EDGE_CURVE ( 'NONE', #87918, #24428, #29980, .T. ) ;
#127010=ORIENTED_EDGE ( 'NONE', *, *, #119044, .F. ) ;
#127011=CARTESIAN_POINT ( 'NONE',  ( -7.050000000000013145, 2.500000000000000000, 2.265063509461097357 ) ) ;
#127012=CARTESIAN_POINT ( 'NONE',  ( 7.099999999999928590, 12.50000000000000000, -5.022947341949754119 ) ) ;
#127013=ADVANCED_FACE ( 'NONE', ( #115787 ), #27808, .T. ) ;
#127014=AXIS2_PLACEMENT_3D ( 'NONE', #100962, #51250, #118025 ) ;
#127015=CARTESIAN_POINT ( 'NONE',  ( 12.89999999999990088, 2.500000000000000000, -4.330127018922201643 ) ) ;
#127016=AXIS2_PLACEMENT_3D ( 'NONE', #90000, #120127, #107722 ) ;
#127017=DIRECTION ( 'NONE',  ( -0.000000000000000000, -1.000000000000000000, -0.000000000000000000 ) ) ;
#127018=ORIENTED_EDGE ( 'NONE', *, *, #120394, .F. ) ;
#127019=DIRECTION ( 'NONE',  ( -0.000000000000000000, 1.000000000000000000, -0.000000000000000000 ) ) ;
#127020=ADVANCED_FACE ( 'NONE', ( #38550 ), #34088, .T. ) ;
#127021=AXIS2_PLACEMENT_3D ( 'NONE', #43891, #54973, #123695 ) ;
#127022=AXIS2_PLACEMENT_3D ( 'NONE', #5258, #35384, #55657 ) ;
#127023=EDGE_CURVE ( 'NONE', #117617, #24882, #67298, .T. ) ;
#127024=DIRECTION ( 'NONE',  ( -0.000000000000000000, 1.000000000000000000, -0.000000000000000000 ) ) ;
#127025=VERTEX_POINT ( 'NONE', #17576 ) ;
#127026=DIRECTION ( 'NONE',  ( -0.000000000000000000, -1.000000000000000000, -0.000000000000000000 ) ) ;
#127027=CIRCLE ( 'NONE', #89449, 0.1000000000000000472 ) ;
#127028=ADVANCED_FACE ( 'NONE', ( #128865 ), #61282, .T. ) ;
#127029=CARTESIAN_POINT ( 'NONE',  ( -8.350000000000013856, 12.50000000000000000, -7.188010851410848723 ) ) ;
#127030=FACE_BOUND ( 'NONE', #68042, .T. ) ;
#127031=ADVANCED_FACE ( 'NONE', ( #57525 ), #11075, .T. ) ;
#127032=DIRECTION ( 'NONE',  ( 0.000000000000000000, 0.000000000000000000, 1.000000000000000000 ) ) ;
#127033=VECTOR ( 'NONE', #21820, 1000.000000000000000 ) ;
#127034=AXIS2_PLACEMENT_3D ( 'NONE', #97682, #55829, #66292 ) ;
#127035=EDGE_LOOP ( 'NONE', ( #64154, #83921, #73055, #85120 ) ) ;
#127036=CARTESIAN_POINT ( 'NONE',  ( -5.850000000000018296, 2.500000000000000000, 1.572243186433545548 ) ) ;
#127037=ORIENTED_EDGE ( 'NONE', *, *, #74662, .F. ) ;
#127039=VERTEX_POINT ( 'NONE', #7759 ) ;
#127040=CARTESIAN_POINT ( 'NONE',  ( -5.400000000000023448, 2.500000000000000000, -5.022947341949754119 ) ) ;
#127042=EDGE_LOOP ( 'NONE', ( #115641, #21487, #63976, #30578 ) ) ;
#127043=LINE ( 'NONE', #20941, #36561 ) ;
#127044=CARTESIAN_POINT ( 'NONE',  ( -8.550000000000013145, 12.50000000000000000, -6.776507416713036136 ) ) ;
#127045=DIRECTION ( 'NONE',  ( -0.000000000000000000, -1.000000000000000000, -0.000000000000000000 ) ) ;
#127047=ORIENTED_EDGE ( 'NONE', *, *, #106401, .F. ) ;
#127048=FACE_OUTER_BOUND ( 'NONE', #73287, .T. ) ;
#127049=CARTESIAN_POINT ( 'NONE',  ( -13.09999999999999254, 2.500000000000000000, -4.576537180435974683 ) ) ;
#127050=CARTESIAN_POINT ( 'NONE',  ( -3.350000000000032507, 2.500000000000000000, -6.495190528383302464 ) ) ;
#127051=CARTESIAN_POINT ( 'NONE',  ( 16.55712542098053319, 0.2763552092525495829, -6.093697598455521280 ) ) ;
#127052=ORIENTED_EDGE ( 'NONE', *, *, #639, .T. ) ;
#127053=DIRECTION ( 'NONE',  ( 0.000000000000000000, -0.000000000000000000, 1.000000000000000000 ) ) ;
#127054=ORIENTED_EDGE ( 'NONE', *, *, #7565, .F. ) ;
#127055=FACE_OUTER_BOUND ( 'NONE', #80481, .T. ) ;
#127056=CARTESIAN_POINT ( 'NONE',  ( -12.09999999999999432, 2.500000000000000000, 5.022947341949748790 ) ) ;
#127057=ORIENTED_EDGE ( 'NONE', *, *, #84900, .T. ) ;
#127058=CARTESIAN_POINT ( 'NONE',  ( -7.700000000000014388, 12.50000000000000000, -4.676537180435977881 ) ) ;
#127059=PLANE ( 'NONE',  #68241 ) ;
#127060=ADVANCED_FACE ( 'NONE', ( #96776 ), #19494, .T. ) ;
#127061=DIRECTION ( 'NONE',  ( 0.000000000000000000, 0.000000000000000000, 1.000000000000000000 ) ) ;
#127062=AXIS2_PLACEMENT_3D ( 'NONE', #85906, #125837, #66282 ) ;
#127063=DIRECTION ( 'NONE',  ( 0.000000000000000000, -0.000000000000000000, 1.000000000000000000 ) ) ;
#127064=EDGE_LOOP ( 'NONE', ( #94224, #43696 ) ) ;
#127065=DIRECTION ( 'NONE',  ( 0.000000000000000000, 1.000000000000000000, 0.000000000000000000 ) ) ;
#127066=EDGE_CURVE ( 'NONE', #124332, #28942, #109385, .T. ) ;
#127067=CARTESIAN_POINT ( 'NONE',  ( 5.399999999999936406, 12.50000000000000000, -3.637306695894650055 ) ) ;
#127069=CARTESIAN_POINT ( 'NONE',  ( -8.350000000000012079, 2.500000000000000000, 2.857883832488649301 ) ) ;
#127070=DIRECTION ( 'NONE',  ( 0.000000000000000000, -0.9999939076577903929, 0.003490651415223739937 ) ) ;
#127071=AXIS2_PLACEMENT_3D ( 'NONE', #127896, #78162, #28414 ) ;
#127072=ORIENTED_EDGE ( 'NONE', *, *, #86154, .F. ) ;
#127073=AXIS2_PLACEMENT_3D ( 'NONE', #696, #90358, #11807 ) ;
#127074=CONICAL_SURFACE ( 'NONE', #123145, 0.1000000000000002554, 0.003490658503988666988 ) ;
#127075=ORIENTED_EDGE ( 'NONE', *, *, #111446, .T. ) ;
#127076=DIRECTION ( 'NONE',  ( -0.000000000000000000, 1.000000000000000000, -0.000000000000000000 ) ) ;
#127077=EDGE_LOOP ( 'NONE', ( #76267, #88518, #129112, #14595 ) ) ;
#127078=DIRECTION ( 'NONE',  ( 0.000000000000000000, 0.000000000000000000, 1.000000000000000000 ) ) ;
#127079=EDGE_LOOP ( 'NONE', ( #90658, #32491, #65977, #86208 ) ) ;
#127080=ORIENTED_EDGE ( 'NONE', *, *, #79153, .F. ) ;
#127081=ORIENTED_EDGE ( 'NONE', *, *, #45469, .F. ) ;
#127082=CARTESIAN_POINT ( 'NONE',  ( -0.8500000000000390576, 12.50000000000000000, -6.495190528383302464 ) ) ;
#127083=VECTOR ( 'NONE', #85177, 1000.000000000000000 ) ;
#127084=DIRECTION ( 'NONE',  ( 0.000000000000000000, 1.000000000000000000, 0.000000000000000000 ) ) ;
#127085=DIRECTION ( 'NONE',  ( 0.000000000000000000, 0.000000000000000000, -1.000000000000000000 ) ) ;
#127087=DIRECTION ( 'NONE',  ( -0.000000000000000000, -1.000000000000000000, -0.000000000000000000 ) ) ;
#127088=LINE ( 'NONE', #37421, #96109 ) ;
#127090=CIRCLE ( 'NONE', #104092, 0.09999999999999982514 ) ;
#127091=VERTEX_POINT ( 'NONE', #9707 ) ;
#127092=PLANE ( 'NONE',  #95751 ) ;
#127093=VERTEX_POINT ( 'NONE', #87609 ) ;
#127094=AXIS2_PLACEMENT_3D ( 'NONE', #12526, #82583, #122499 ) ;
#127095=EDGE_LOOP ( 'NONE', ( #88157, #107369 ) ) ;
#127096=EDGE_LOOP ( 'NONE', ( #8553, #81955, #83840, #41079 ) ) ;
#127097=ORIENTED_EDGE ( 'NONE', *, *, #74116, .T. ) ;
#127098=CONICAL_SURFACE ( 'NONE', #60203, 0.09999999999999982514, 0.003490658503988666988 ) ;
#127099=DIRECTION ( 'NONE',  ( -0.000000000000000000, -1.000000000000000000, -0.000000000000000000 ) ) ;
#127100=EDGE_LOOP ( 'NONE', ( #18003, #81535, #61690, #34424 ) ) ;
#127101=EDGE_LOOP ( 'NONE', ( #73071, #42332 ) ) ;
#127102=CONICAL_SURFACE ( 'NONE', #87360, 0.09999999999999982514, 0.003490658503988666988 ) ;
#127103=CIRCLE ( 'NONE', #22555, 0.1000000000000002554 ) ;
#127104=ADVANCED_FACE ( 'NONE', ( #58181 ), #77781, .T. ) ;
#127105=DIRECTION ( 'NONE',  ( 0.000000000000000000, -0.000000000000000000, 1.000000000000000000 ) ) ;
#127106=CARTESIAN_POINT ( 'NONE',  ( 2.499999999999981792, 2.500000000000000000, 4.330127018922196314 ) ) ;
#127107=AXIS2_PLACEMENT_3D ( 'NONE', #21873, #120702, #2860 ) ;
#127108=LINE ( 'NONE', #37440, #63170 ) ;
#127109=DIRECTION ( 'NONE',  ( 0.000000000000000000, 0.000000000000000000, 1.000000000000000000 ) ) ;
#127110=CARTESIAN_POINT ( 'NONE',  ( -10.45000000000000107, 12.50000000000000000, 6.430097255199259010 ) ) ;
#127111=ORIENTED_EDGE ( 'NONE', *, *, #34273, .F. ) ;
#127112=AXIS2_PLACEMENT_3D ( 'NONE', #23057, #33534, #74089 ) ;
#127113=CARTESIAN_POINT ( 'NONE',  ( 2.299999999999946976, 2.500000000000000000, 4.776537180435972196 ) ) ;
#127114=AXIS2_PLACEMENT_3D ( 'NONE', #65707, #123976, #75517 ) ;
#127115=EDGE_LOOP ( 'NONE', ( #39105, #127536 ) ) ;
#127116=AXIS2_PLACEMENT_3D ( 'NONE', #9781, #88993, #89639 ) ;
#127117=CARTESIAN_POINT ( 'NONE',  ( 2.500000000000002220, 1.500000000000000444, -9.999999999999998224 ) ) ;
#127118=EDGE_LOOP ( 'NONE', ( #35714, #111055 ) ) ;
#127119=DIRECTION ( 'NONE',  ( 0.000000000000000000, 0.000000000000000000, -1.000000000000000000 ) ) ;
#127120=EDGE_LOOP ( 'NONE', ( #32972, #30857, #57037, #38736 ) ) ;
#127121=ADVANCED_FACE ( 'NONE', ( #7109 ), #9022, .T. ) ;
#127122=AXIS2_PLACEMENT_3D ( 'NONE', #46359, #128160, #56810 ) ;
#127123=EDGE_CURVE ( 'NONE', #47068, #77555, #618, .T. ) ;
#127124=EDGE_LOOP ( 'NONE', ( #124535, #96011, #21385, #52093 ) ) ;
#127125=CARTESIAN_POINT ( 'NONE',  ( -1.900000000000034994, 2.500000000000000000, -0.3464101615137783474 ) ) ;
#127126=CARTESIAN_POINT ( 'NONE',  ( 6.899999999999926636, 12.50000000000000000, 0.4115034346978110880 ) ) ;
#127127=CIRCLE ( 'NONE', #66552, 0.1000000000000002554 ) ;
#127128=CONICAL_SURFACE ( 'NONE', #1710, 0.1000000000000002554, 0.003490658503988666988 ) ;
#127129=PLANE ( 'NONE',  #94761 ) ;
#127130=CARTESIAN_POINT ( 'NONE',  ( 3.349999999999943689, 2.500000000000000000, 2.165063509461097713 ) ) ;
#127131=CARTESIAN_POINT ( 'NONE',  ( -13.14999999999999147, 2.500000000000000000, -2.511473670974875727 ) ) ;
#127132=ORIENTED_EDGE ( 'NONE', *, *, #92188, .T. ) ;
#127133=DIRECTION ( 'NONE',  ( 0.000000000000000000, 0.000000000000000000, -1.000000000000000000 ) ) ;
#127134=CARTESIAN_POINT ( 'NONE',  ( -1.050000000000038236, 2.500000000000000000, -6.148780366869526226 ) ) ;
#127135=ADVANCED_FACE ( 'NONE', ( #48340 ), #18870, .T. ) ;
#127136=CARTESIAN_POINT ( 'NONE',  ( 9.399999999999918643, 2.500000000000000000, 0.3464101615137736845 ) ) ;
#127137=DIRECTION ( 'NONE',  ( 0.000000000000000000, -0.000000000000000000, 1.000000000000000000 ) ) ;
#127138=CARTESIAN_POINT ( 'NONE',  ( -1.850000000000033840, 2.500000000000000000, 6.841600689897072485 ) ) ;
#127139=EDGE_LOOP ( 'NONE', ( #42789, #118299 ) ) ;
#127140=ORIENTED_EDGE ( 'NONE', *, *, #88885, .F. ) ;
#127141=LINE ( 'NONE', #59038, #113535 ) ;
#127142=ORIENTED_EDGE ( 'NONE', *, *, #83995, .F. ) ;
#127143=DIRECTION ( 'NONE',  ( -0.000000000000000000, -1.000000000000000000, -0.000000000000000000 ) ) ;
#127144=CARTESIAN_POINT ( 'NONE',  ( 3.949999999999941558, 12.50000000000000000, -6.148780366869526226 ) ) ;
#127145=AXIS2_PLACEMENT_3D ( 'NONE', #3263, #85677, #83753 ) ;
#127146=VECTOR ( 'NONE', #48352, 1000.000000000000000 ) ;
#127147=CIRCLE ( 'NONE', #70698, 0.1000000000000002554 ) ;
#127148=ORIENTED_EDGE ( 'NONE', *, *, #48554, .F. ) ;
#127150=CARTESIAN_POINT ( 'NONE',  ( 7.049999999999928768, 2.500000000000000000, -2.165063509461101710 ) ) ;
#127151=DIRECTION ( 'NONE',  ( -0.000000000000000000, 1.000000000000000000, -0.000000000000000000 ) ) ;
#127152=FACE_OUTER_BOUND ( 'NONE', #62521, .T. ) ;
#127153=ORIENTED_EDGE ( 'NONE', *, *, #14231, .F. ) ;
#127155=EDGE_CURVE ( 'NONE', #35157, #37472, #4811, .T. ) ;
#127156=AXIS2_PLACEMENT_3D ( 'NONE', #103264, #22145, #62060 ) ;
#127157=CARTESIAN_POINT ( 'NONE',  ( -5.650000000000023448, 12.50000000000000000, -2.511473670974877948 ) ) ;
#127158=DIRECTION ( 'NONE',  ( 0.000000000000000000, 0.000000000000000000, 1.000000000000000000 ) ) ;
#127159=VERTEX_POINT ( 'NONE', #28061 ) ;
#127160=EDGE_CURVE ( 'NONE', #88991, #29584, #86389, .T. ) ;
#127161=DIRECTION ( 'NONE',  ( -0.000000000000000000, 1.000000000000000000, -0.000000000000000000 ) ) ;
#127162=DIRECTION ( 'NONE',  ( -4.274815082592931898E-19, -0.9999939076577903929, -0.003490651415223739937 ) ) ;
#127163=CIRCLE ( 'NONE', #91642, 0.06509327318403745899 ) ;
#127164=EDGE_CURVE ( 'NONE', #61588, #2220, #111428, .T. ) ;
#127165=CARTESIAN_POINT ( 'NONE',  ( -5.800000000000022027, 2.500000000000000000, -4.330127018922201643 ) ) ;
#127166=CIRCLE ( 'NONE', #60283, 0.06509327318403741736 ) ;
#127167=ORIENTED_EDGE ( 'NONE', *, *, #109250, .T. ) ;
#127168=CARTESIAN_POINT ( 'NONE',  ( 11.24999999999994316, 12.50000000000000000, -6.495190528383302464 ) ) ;
#127170=ADVANCED_FACE ( 'NONE', ( #109175 ), #69671, .T. ) ;
#127171=VERTEX_POINT ( 'NONE', #90172 ) ;
#127172=DIRECTION ( 'NONE',  ( -0.000000000000000000, 1.000000000000000000, -0.000000000000000000 ) ) ;
#127173=CARTESIAN_POINT ( 'NONE',  ( 9.149999999999915090, 12.50000000000000000, -2.165063509461101710 ) ) ;
#127174=ADVANCED_FACE ( 'NONE', ( #20169 ), #128175, .T. ) ;
#127175=ADVANCED_FACE ( 'NONE', ( #80392 ), #98923, .T. ) ;
#127176=CARTESIAN_POINT ( 'NONE',  ( 6.249999999999928946, 2.500000000000000000, 2.757883832488649656 ) ) ;
#127177=VERTEX_POINT ( 'NONE', #60743 ) ;
#127178=AXIS2_PLACEMENT_3D ( 'NONE', #54912, #13039, #25437 ) ;
#127179=DIRECTION ( 'NONE',  ( 0.000000000000000000, 0.000000000000000000, 1.000000000000000000 ) ) ;
#127180=ADVANCED_FACE ( 'NONE', ( #2442 ), #60117, .T. ) ;
#127181=PLANE ( 'NONE',  #101785 ) ;
#127182=AXIS2_PLACEMENT_3D ( 'NONE', #124551, #25050, #3475 ) ;
#127183=VERTEX_POINT ( 'NONE', #52213 ) ;
#127184=CARTESIAN_POINT ( 'NONE',  ( 12.09999999999990195, 12.50000000000000000, -2.276824562219559311E-15 ) ) ;
#127185=ORIENTED_EDGE ( 'NONE', *, *, #15711, .T. ) ;
#127186=EDGE_CURVE ( 'NONE', #104669, #43749, #103128, .T. ) ;
#127187=LINE ( 'NONE', #6714, #74514 ) ;
#127188=AXIS2_PLACEMENT_3D ( 'NONE', #119688, #90221, #92833 ) ;
#127189=ORIENTED_EDGE ( 'NONE', *, *, #61515, .F. ) ;
#127190=CARTESIAN_POINT ( 'NONE',  ( -3.100000000000028511, 12.50000000000000000, -3.918623584224389056 ) ) ;
#127191=FACE_OUTER_BOUND ( 'NONE', #105684, .T. ) ;
#127193=ORIENTED_EDGE ( 'NONE', *, *, #9778, .T. ) ;
#127194=CARTESIAN_POINT ( 'NONE',  ( 5.649999999999936406, 2.500000000000000000, -6.741600689897077281 ) ) ;
#127195=DIRECTION ( 'NONE',  ( 0.000000000000000000, 1.000000000000000000, 0.000000000000000000 ) ) ;
#127196=VERTEX_POINT ( 'NONE', #92786 ) ;
#127197=DIRECTION ( 'NONE',  ( -4.274815082592931898E-19, -0.9999939076577903929, -0.003490651415223739937 ) ) ;
#127198=CARTESIAN_POINT ( 'NONE',  ( -2.100000000000033840, 12.50000000000000000, 3.637306695894644726 ) ) ;
#127199=VECTOR ( 'NONE', #34761, 1000.000000000000000 ) ;
#127200=CARTESIAN_POINT ( 'NONE',  ( 5.649999999999936406, 12.50000000000000000, -6.841600689897077814 ) ) ;
#127201=DIRECTION ( 'NONE',  ( -0.000000000000000000, 1.000000000000000000, -0.000000000000000000 ) ) ;
#127202=CARTESIAN_POINT ( 'NONE',  ( -5.800000000000018474, 12.50000000000000000, 4.265033745738159077 ) ) ;
#127203=CARTESIAN_POINT ( 'NONE',  ( -3.550000000000027356, 12.50000000000000000, 1.818653347947321475 ) ) ;
#127204=ORIENTED_EDGE ( 'NONE', *, *, #112665, .F. ) ;
#127205=ORIENTED_EDGE ( 'NONE', *, *, #54700, .F. ) ;
#127206=VERTEX_POINT ( 'NONE', #82323 ) ;
#127207=ORIENTED_EDGE ( 'NONE', *, *, #17796, .T. ) ;
#127208=PLANE ( 'NONE',  #45419 ) ;
#127209=CARTESIAN_POINT ( 'NONE',  ( 4.149999999999939959, 2.500000000000000000, -2.065063509461102065 ) ) ;
#127210=CARTESIAN_POINT ( 'NONE',  ( -10.60000000000000142, 2.500000000000000000, 3.883716857408421319 ) ) ;
#127211=VECTOR ( 'NONE', #31257, 1000.000000000000000 ) ;
#127212=EDGE_LOOP ( 'NONE', ( #51492, #120156 ) ) ;
#127213=FACE_BOUND ( 'NONE', #77444, .T. ) ;
#127214=FACE_OUTER_BOUND ( 'NONE', #81408, .T. ) ;
#127215=CARTESIAN_POINT ( 'NONE',  ( 3.349999999999943689, 2.500000000000000000, 1.372243186433545370 ) ) ;
#127216=DIRECTION ( 'NONE',  ( 0.000000000000000000, -0.000000000000000000, 1.000000000000000000 ) ) ;
#127217=CONICAL_SURFACE ( 'NONE', #14314, 0.1000000000000002554, 0.003490658503988666988 ) ;
#127218=CONICAL_SURFACE ( 'NONE', #39500, 0.09999999999999982514, 0.003490658503988666988 ) ;
#127219=ADVANCED_FACE ( 'NONE', ( #511 ), #61393, .T. ) ;
#127220=DIRECTION ( 'NONE',  ( 0.000000000000000000, -0.9999939076577903929, 0.003490651415223739937 ) ) ;
#127221=DIRECTION ( 'NONE',  ( 0.000000000000000000, 0.000000000000000000, -1.000000000000000000 ) ) ;
#127222=LINE ( 'NONE', #87902, #81049 ) ;
#127223=DIRECTION ( 'NONE',  ( 0.000000000000000000, -0.9999939076577903929, 0.003490651415223739937 ) ) ;
#127224=DIRECTION ( 'NONE',  ( 0.000000000000000000, 0.000000000000000000, 1.000000000000000000 ) ) ;
#127225=CARTESIAN_POINT ( 'NONE',  ( -5.200000000000020606, 2.500000000000000000, 3.883716857408421319 ) ) ;
#127226=DIRECTION ( 'NONE',  ( 0.000000000000000000, 0.000000000000000000, 1.000000000000000000 ) ) ;
#127227=ADVANCED_FACE ( 'NONE', ( #22770 ), #62686, .T. ) ;
#127228=ORIENTED_EDGE ( 'NONE', *, *, #78571, .T. ) ;
#127229=ORIENTED_EDGE ( 'NONE', *, *, #6445, .T. ) ;
#127230=ORIENTED_EDGE ( 'NONE', *, *, #39169, .T. ) ;
#127231=ORIENTED_EDGE ( 'NONE', *, *, #70563, .T. ) ;
#127232=DIRECTION ( 'NONE',  ( 0.000000000000000000, 0.000000000000000000, 1.000000000000000000 ) ) ;
#127233=AXIS2_PLACEMENT_3D ( 'NONE', #52328, #105299, #92917 ) ;
#127234=DIRECTION ( 'NONE',  ( -0.000000000000000000, 1.000000000000000000, -0.000000000000000000 ) ) ;
#127235=ORIENTED_EDGE ( 'NONE', *, *, #79401, .T. ) ;
#127236=EDGE_LOOP ( 'NONE', ( #24999, #106929 ) ) ;
#127237=ORIENTED_EDGE ( 'NONE', *, *, #116091, .T. ) ;
#127238=DIRECTION ( 'NONE',  ( 0.000000000000000000, -0.9999939076577903929, 0.003490651415223739937 ) ) ;
#127239=AXIS2_PLACEMENT_3D ( 'NONE', #70286, #89274, #79467 ) ;
#127240=DIRECTION ( 'NONE',  ( -0.000000000000000000, -1.000000000000000000, -0.000000000000000000 ) ) ;
#127241=AXIS2_PLACEMENT_3D ( 'NONE', #109862, #108565, #18884 ) ;
#127242=CARTESIAN_POINT ( 'NONE',  ( 9.599999999999914380, 2.500000000000000000, -4.922947341949753586 ) ) ;
#127245=CARTESIAN_POINT ( 'NONE',  ( 11.04999999999991189, 12.50000000000000000, 6.213873640053559022 ) ) ;
#127246=EDGE_LOOP ( 'NONE', ( #22324, #11274 ) ) ;
#127247=DIRECTION ( 'NONE',  ( -0.000000000000000000, 1.000000000000000000, -0.000000000000000000 ) ) ;
#127248=ORIENTED_EDGE ( 'NONE', *, *, #81897, .T. ) ;
#127249=CIRCLE ( 'NONE', #129417, 0.06509327318403745899 ) ;
#127250=VERTEX_POINT ( 'NONE', #122250 ) ;
#127251=ORIENTED_EDGE ( 'NONE', *, *, #78306, .F. ) ;
#127252=CIRCLE ( 'NONE', #87508, 0.06509327318403745899 ) ;
#127253=CARTESIAN_POINT ( 'NONE',  ( 9.149999999999916866, 2.500000000000000000, 5.802370205355744659 ) ) ;
#127255=ORIENTED_EDGE ( 'NONE', *, *, #87568, .T. ) ;
#127256=CIRCLE ( 'NONE', #31205, 0.06509327318403745899 ) ;
#127257=CARTESIAN_POINT ( 'NONE',  ( 1.049999999999953637, 2.500000000000000000, -1.818653347947326138 ) ) ;
#127258=AXIS2_PLACEMENT_3D ( 'NONE', #87024, #26826, #106029 ) ;
#127259=ADVANCED_FACE ( 'NONE', ( #62040 ), #32598, .T. ) ;
#127260=CARTESIAN_POINT ( 'NONE',  ( 11.84999999999990727, 2.500000000000000000, -1.818653347947326138 ) ) ;
#127261=FACE_OUTER_BOUND ( 'NONE', #47916, .T. ) ;
#127263=DIRECTION ( 'NONE',  ( 0.000000000000000000, 0.000000000000000000, 1.000000000000000000 ) ) ;
#127264=EDGE_LOOP ( 'NONE', ( #24201, #57644, #125348, #76677 ) ) ;
#127265=DIRECTION ( 'NONE',  ( -0.000000000000000000, 1.000000000000000000, -0.000000000000000000 ) ) ;
#127266=AXIS2_PLACEMENT_3D ( 'NONE', #118996, #79719, #70538 ) ;
#127267=EDGE_CURVE ( 'NONE', #16136, #60318, #88446, .T. ) ;
#127268=ORIENTED_EDGE ( 'NONE', *, *, #3678, .F. ) ;
#127269=CARTESIAN_POINT ( 'NONE',  ( 2.899999999999944844, 2.500000000000000000, 5.122947341949749323 ) ) ;
#127270=ORIENTED_EDGE ( 'NONE', *, *, #106648, .F. ) ;
#127271=CARTESIAN_POINT ( 'NONE',  ( 0.7999999999999612976, 2.500000000000000000, -0.1000000000000001166 ) ) ;
#127272=CARTESIAN_POINT ( 'NONE',  ( -9.600000000000006750, 12.50000000000000000, 3.702399969078682407 ) ) ;
#127273=CIRCLE ( 'NONE', #70815, 0.09999999999999982514 ) ;
#127275=FACE_OUTER_BOUND ( 'NONE', #48632, .T. ) ;
#127276=EDGE_CURVE ( 'NONE', #36888, #95931, #102584, .T. ) ;
#127277=LINE ( 'NONE', #47425, #89571 ) ;
#127278=EDGE_CURVE ( 'NONE', #2822, #91444, #90502, .T. ) ;
#127279=ORIENTED_EDGE ( 'NONE', *, *, #101142, .T. ) ;
#127280=EDGE_CURVE ( 'NONE', #20773, #101675, #107232, .T. ) ;
#127281=CARTESIAN_POINT ( 'NONE',  ( -3.749999999999994671, 2.500000000000000000, -6.495190528383302464 ) ) ;
#127282=ORIENTED_EDGE ( 'NONE', *, *, #21784, .F. ) ;
#127283=ORIENTED_EDGE ( 'NONE', *, *, #47388, .T. ) ;
#127284=CARTESIAN_POINT ( 'NONE',  ( 5.649999999999932854, 12.50000000000000000, 1.818653347947321475 ) ) ;
#127285=DIRECTION ( 'NONE',  ( 0.000000000000000000, -0.000000000000000000, 1.000000000000000000 ) ) ;
#127286=ADVANCED_FACE ( 'NONE', ( #33235 ), #115632, .T. ) ;
#127288=DIRECTION ( 'NONE',  ( -0.000000000000000000, 1.000000000000000000, -0.000000000000000000 ) ) ;
#127289=CIRCLE ( 'NONE', #18609, 0.1000000000000002554 ) ;
#127290=DIRECTION ( 'NONE',  ( 0.000000000000000000, 0.000000000000000000, 1.000000000000000000 ) ) ;
#127291=CARTESIAN_POINT ( 'NONE',  ( 10.64999999999990976, 12.50000000000000000, 1.818653347947321475 ) ) ;
#127293=ORIENTED_EDGE ( 'NONE', *, *, #5632, .T. ) ;
#127294=CARTESIAN_POINT ( 'NONE',  ( 8.749999999999957367, 12.50000000000000000, 2.165063509461097713 ) ) ;
#127295=CARTESIAN_POINT ( 'NONE',  ( 5.649999999999934630, 2.500000000000000000, 6.741600689897071952 ) ) ;
#127296=ORIENTED_EDGE ( 'NONE', *, *, #50853, .F. ) ;
#127297=AXIS2_PLACEMENT_3D ( 'NONE', #112641, #13775, #2656 ) ;
#127298=VECTOR ( 'NONE', #14297, 1000.000000000000000 ) ;
#127299=CIRCLE ( 'NONE', #14403, 0.06509327318403745899 ) ;
#127300=PLANE ( 'NONE',  #24285 ) ;
#127302=CARTESIAN_POINT ( 'NONE',  ( 1.449999999999949551, 12.50000000000000000, 6.906693963081109722 ) ) ;
#127303=CARTESIAN_POINT ( 'NONE',  ( 0.5999999999999547917, 2.500000000000000000, 3.983716857408420076 ) ) ;
#127304=CARTESIAN_POINT ( 'NONE',  ( -9.400000000000007461, 2.500000000000000000, 0.4464101615137735513 ) ) ;
#127305=ORIENTED_EDGE ( 'NONE', *, *, #4766, .T. ) ;
#127306=CIRCLE ( 'NONE', #66737, 0.06509327318403745899 ) ;
#127307=CARTESIAN_POINT ( 'NONE',  ( -3.750000000000027534, 2.500000000000000000, -1.472243186433550122 ) ) ;
#127309=ORIENTED_EDGE ( 'NONE', *, *, #4615, .F. ) ;
#127310=EDGE_CURVE ( 'NONE', #73222, #99644, #80147, .T. ) ;
#127311=FACE_OUTER_BOUND ( 'NONE', #71811, .T. ) ;
#127312=VERTEX_POINT ( 'NONE', #71196 ) ;
#127313=EDGE_LOOP ( 'NONE', ( #45710, #29462, #1970, #123839 ) ) ;
#127314=DIRECTION ( 'NONE',  ( 0.000000000000000000, 0.000000000000000000, 1.000000000000000000 ) ) ;
#127315=ADVANCED_FACE ( 'NONE', ( #111098 ), #36347, .T. ) ;
#127316=CIRCLE ( 'NONE', #24903, 0.1000000000000000472 ) ;
#127317=EDGE_CURVE ( 'NONE', #84067, #83209, #91483, .T. ) ;
#127318=ORIENTED_EDGE ( 'NONE', *, *, #49921, .F. ) ;
#127319=DIRECTION ( 'NONE',  ( -4.274815082592931898E-19, -0.9999939076577903929, -0.003490651415223739937 ) ) ;
#127320=FACE_OUTER_BOUND ( 'NONE', #15728, .T. ) ;
#127321=ADVANCED_FACE ( 'NONE', ( #65885 ), #103888, .T. ) ;
#127322=EDGE_CURVE ( 'NONE', #12969, #59349, #95362, .T. ) ;
#127323=DIRECTION ( 'NONE',  ( 0.000000000000000000, 0.000000000000000000, 1.000000000000000000 ) ) ;
#127324=EDGE_LOOP ( 'NONE', ( #116920, #101533 ) ) ;
#127325=VECTOR ( 'NONE', #69315, 1000.000000000000000 ) ;
#127326=FACE_BOUND ( 'NONE', #129441, .T. ) ;
#127327=CONICAL_SURFACE ( 'NONE', #87590, 0.1000000000000002554, 0.003490658503988666988 ) ;
#127328=EDGE_CURVE ( 'NONE', #2568, #28423, #96951, .T. ) ;
#127329=DIRECTION ( 'NONE',  ( 0.000000000000000000, 0.000000000000000000, -1.000000000000000000 ) ) ;
#127330=ORIENTED_EDGE ( 'NONE', *, *, #17763, .T. ) ;
#127331=CARTESIAN_POINT ( 'NONE',  ( 11.64999999999990443, 12.50000000000000000, -5.867463478539787225 ) ) ;
#127332=CARTESIAN_POINT ( 'NONE',  ( -3.100000000000028511, 2.500000000000000000, -4.676537180435977881 ) ) ;
#127333=CIRCLE ( 'NONE', #72951, 0.06509327318403745899 ) ;
#127334=EDGE_LOOP ( 'NONE', ( #10923, #57065, #88711, #100480 ) ) ;
#127335=AXIS2_PLACEMENT_3D ( 'NONE', #6465, #86341, #108574 ) ;
#127336=ADVANCED_FACE ( 'NONE', ( #23376 ), #128278, .T. ) ;
#127337=AXIS2_PLACEMENT_3D ( 'NONE', #3276, #34024, #22293 ) ;
#127338=EDGE_CURVE ( 'NONE', #46960, #96127, #75698, .T. ) ;
#127339=ORIENTED_EDGE ( 'NONE', *, *, #23218, .F. ) ;
#127340=ORIENTED_EDGE ( 'NONE', *, *, #26339, .T. ) ;
#127341=CARTESIAN_POINT ( 'NONE',  ( -2.700000000000030820, 2.500000000000000000, -3.983716857408426293 ) ) ;
#127342=CARTESIAN_POINT ( 'NONE',  ( -12.49999999999995914, 2.500000000000000000, -4.330127018922198978 ) ) ;
#127343=DIRECTION ( 'NONE',  ( 0.000000000000000000, 0.000000000000000000, -1.000000000000000000 ) ) ;
#127344=FACE_BOUND ( 'NONE', #1781, .T. ) ;
#127345=ORIENTED_EDGE ( 'NONE', *, *, #104113, .F. ) ;
#127346=CARTESIAN_POINT ( 'NONE',  ( -11.44999999999999751, 2.500000000000000000, 1.818653347947321475 ) ) ;
#127347=CARTESIAN_POINT ( 'NONE',  ( 3.149999999999944400, 12.50000000000000000, 1.883746621131358934 ) ) ;
#127348=ORIENTED_EDGE ( 'NONE', *, *, #49749, .T. ) ;
#127349=AXIS2_PLACEMENT_3D ( 'NONE', #60796, #124874, #25357 ) ;
#127350=DIRECTION ( 'NONE',  ( 0.000000000000000000, 0.000000000000000000, 1.000000000000000000 ) ) ;
#127351=LINE ( 'NONE', #27195, #71671 ) ;
#127352=CARTESIAN_POINT ( 'NONE',  ( -2.100000000000033396, 12.50000000000000000, -3.637306695894650055 ) ) ;
#127353=DIRECTION ( 'NONE',  ( -0.000000000000000000, -1.000000000000000000, -0.000000000000000000 ) ) ;
#127354=ADVANCED_FACE ( 'NONE', ( #14196 ), #69770, .T. ) ;
#127355=PLANE ( 'NONE',  #44017 ) ;
#127356=ORIENTED_EDGE ( 'NONE', *, *, #115744, .T. ) ;
#127357=ORIENTED_EDGE ( 'NONE', *, *, #30283, .F. ) ;
#127358=ORIENTED_EDGE ( 'NONE', *, *, #89105, .T. ) ;
#127360=ORIENTED_EDGE ( 'NONE', *, *, #21073, .T. ) ;
#127361=AXIS2_PLACEMENT_3D ( 'NONE', #115445, #47382, #65059 ) ;
#127362=CARTESIAN_POINT ( 'NONE',  ( 11.44999999999990692, 2.500000000000000000, 1.818653347947321475 ) ) ;
#127363=DIRECTION ( 'NONE',  ( -4.274815082592931898E-19, -0.9999939076577903929, -0.003490651415223739937 ) ) ;
#127364=ORIENTED_EDGE ( 'NONE', *, *, #61971, .F. ) ;
#127365=FACE_BOUND ( 'NONE', #58083, .T. ) ;
#127366=CARTESIAN_POINT ( 'NONE',  ( 6.249999999999930722, 2.500000000000000000, -1.372243186433550033 ) ) ;
#127367=DIRECTION ( 'NONE',  ( 0.000000000000000000, 0.000000000000000000, 1.000000000000000000 ) ) ;
#127369=DIRECTION ( 'NONE',  ( 0.000000000000000000, 1.000000000000000000, 0.000000000000000000 ) ) ;
#127370=FACE_OUTER_BOUND ( 'NONE', #29767, .T. ) ;
#127371=VERTEX_POINT ( 'NONE', #25978 ) ;
#127372=CONICAL_SURFACE ( 'NONE', #75132, 0.1000000000000000056, 0.003490658503988666988 ) ;
#127373=CARTESIAN_POINT ( 'NONE',  ( 17.50982737979214932, -2.500000000000000000, 4.074750942089497840 ) ) ;
#127375=ADVANCED_FACE ( 'NONE', ( #124822 ), #40550, .T. ) ;
#127376=VERTEX_POINT ( 'NONE', #36457 ) ;
#127377=ORIENTED_EDGE ( 'NONE', *, *, #120908, .T. ) ;
#127378=DIRECTION ( 'NONE',  ( 0.000000000000000000, 1.000000000000000000, 0.000000000000000000 ) ) ;
#127379=DIRECTION ( 'NONE',  ( 0.000000000000000000, 1.000000000000000000, 0.000000000000000000 ) ) ;
#127380=CARTESIAN_POINT ( 'NONE',  ( -10.85000000000000142, 12.50000000000000000, -2.165063509461097713 ) ) ;
#127381=AXIS2_PLACEMENT_3D ( 'NONE', #79434, #81987, #70891 ) ;
#127382=ORIENTED_EDGE ( 'NONE', *, *, #65797, .T. ) ;
#127383=CARTESIAN_POINT ( 'NONE',  ( 15.40649769424558180, 2.500000000000000444, -5.817321162632842935 ) ) ;
#127384=DIRECTION ( 'NONE',  ( 0.000000000000000000, 0.000000000000000000, 1.000000000000000000 ) ) ;
#127385=CONICAL_SURFACE ( 'NONE', #54224, 0.1000000000000002554, 0.003490658503988666988 ) ;
#127386=CARTESIAN_POINT ( 'NONE',  ( -10.65000000000000391, 12.50000000000000000, -1.818653347947322141 ) ) ;
#127387=CONICAL_SURFACE ( 'NONE', #31246, 0.1000000000000000472, 0.003490658503988666988 ) ;
#127389=CARTESIAN_POINT ( 'NONE',  ( 12.69999999999990337, 2.500000000000000000, 3.983716857408420076 ) ) ;
#127390=DIRECTION ( 'NONE',  ( 0.000000000000000000, 0.000000000000000000, 1.000000000000000000 ) ) ;
#127391=AXIS2_PLACEMENT_3D ( 'NONE', #76327, #28519, #88042 ) ;
#127392=DIRECTION ( 'NONE',  ( 0.000000000000000000, -0.9999939076577903929, 0.003490651415223739937 ) ) ;
#127393=EDGE_LOOP ( 'NONE', ( #60705, #69855, #22132, #126608 ) ) ;
#127394=CARTESIAN_POINT ( 'NONE',  ( -14.99999999999998401, 2.500000000000000000, 0.5928203230275517210 ) ) ;
#127395=CONICAL_SURFACE ( 'NONE', #129568, 0.1000000000000002554, 0.003490658503988666988 ) ;
#127396=ORIENTED_EDGE ( 'NONE', *, *, #102182, .T. ) ;
#127397=ORIENTED_EDGE ( 'NONE', *, *, #94189, .F. ) ;
#127398=FACE_OUTER_BOUND ( 'NONE', #124557, .T. ) ;
#127399=DIRECTION ( 'NONE',  ( -0.000000000000000000, -1.000000000000000000, -0.000000000000000000 ) ) ;
#127401=ORIENTED_EDGE ( 'NONE', *, *, #57417, .T. ) ;
#127402=ORIENTED_EDGE ( 'NONE', *, *, #25632, .T. ) ;
#127403=CARTESIAN_POINT ( 'NONE',  ( 3.149999999999946176, 12.50000000000000000, -6.841600689897077814 ) ) ;
#127404=DIRECTION ( 'NONE',  ( 0.000000000000000000, 0.000000000000000000, 1.000000000000000000 ) ) ;
#127405=DIRECTION ( 'NONE',  ( 0.000000000000000000, 0.000000000000000000, -1.000000000000000000 ) ) ;
#127406=ORIENTED_EDGE ( 'NONE', *, *, #47768, .T. ) ;
#127407=EDGE_LOOP ( 'NONE', ( #22939, #62012, #65838, #38594 ) ) ;
#127408=DIRECTION ( 'NONE',  ( 0.000000000000000000, 0.000000000000000000, -1.000000000000000000 ) ) ;
#127409=EDGE_LOOP ( 'NONE', ( #33561, #102509, #123231, #112514 ) ) ;
#127410=CARTESIAN_POINT ( 'NONE',  ( -12.04999999999999716, 12.50000000000000000, -2.165063509461097713 ) ) ;
#127411=CONICAL_SURFACE ( 'NONE', #10331, 0.1000000000000002554, 0.003490658503988666988 ) ;
#127412=ADVANCED_FACE ( 'NONE', ( #33850 ), #24046, .T. ) ;
#127413=AXIS2_PLACEMENT_3D ( 'NONE', #1214, #32645, #120358 ) ;
#127414=DIRECTION ( 'NONE',  ( -0.000000000000000000, 1.000000000000000000, -0.000000000000000000 ) ) ;
#127415=ORIENTED_EDGE ( 'NONE', *, *, #19270, .F. ) ;
#127416=CARTESIAN_POINT ( 'NONE',  ( 2.499999999999983569, 12.50000000000000000, -4.395220292106239768 ) ) ;
#127417=LINE ( 'NONE', #46265, #52490 ) ;
#127419=ADVANCED_FACE ( 'NONE', ( #113709 ), #54144, .T. ) ;
#127420=CARTESIAN_POINT ( 'NONE',  ( 11.04999999999990834, 2.500000000000000000, 1.718653347947321386 ) ) ;
#127421=EDGE_CURVE ( 'NONE', #11702, #14788, #13318, .T. ) ;
#127422=CONICAL_SURFACE ( 'NONE', #2011, 0.1000000000000002554, 0.003490658503988666988 ) ;
#127423=ORIENTED_EDGE ( 'NONE', *, *, #47504, .T. ) ;
#127424=AXIS2_PLACEMENT_3D ( 'NONE', #4387, #86838, #98574 ) ;
#127425=CARTESIAN_POINT ( 'NONE',  ( -8.550000000000014921, 2.500000000000000000, -6.148780366869520897 ) ) ;
#127426=ADVANCED_FACE ( 'NONE', ( #46245 ), #13557, .T. ) ;
#127428=ADVANCED_FACE ( 'NONE', ( #4362 ), #99014, .T. ) ;
#127429=VERTEX_POINT ( 'NONE', #124167 ) ;
#127430=ADVANCED_FACE ( 'NONE', ( #35164 ), #90596, .T. ) ;
#127431=LINE ( 'NONE', #69134, #45801 ) ;
#127432=CARTESIAN_POINT ( 'NONE',  ( -12.49999999999999467, 2.500000000000000000, 0.6928203230275535862 ) ) ;
#127433=EDGE_CURVE ( 'NONE', #120216, #70218, #103218, .T. ) ;
#127434=CARTESIAN_POINT ( 'NONE',  ( 15.59999999999988951, 12.50000000000000000, 0.3464101615137735735 ) ) ;
#127435=EDGE_CURVE ( 'NONE', #119776, #92740, #34189, .T. ) ;
#127436=CARTESIAN_POINT ( 'NONE',  ( -6.850000000000013856, 2.500000000000000000, 6.941600689897073018 ) ) ;
#127437=CONICAL_SURFACE ( 'NONE', #93975, 0.1000000000000000472, 0.003490658503988666988 ) ;
#127438=DIRECTION ( 'NONE',  ( 0.000000000000000000, -0.9999939076577903929, 0.003490651415223739937 ) ) ;
#127439=FACE_OUTER_BOUND ( 'NONE', #26203, .T. ) ;
#127440=AXIS2_PLACEMENT_3D ( 'NONE', #40201, #98450, #80121 ) ;
#127441=CIRCLE ( 'NONE', #14544, 0.1000000000000002554 ) ;
#127442=DIRECTION ( 'NONE',  ( 0.000000000000000000, 1.000000000000000000, 0.000000000000000000 ) ) ;
#127443=DIRECTION ( 'NONE',  ( 0.000000000000000000, 1.000000000000000000, 0.000000000000000000 ) ) ;
#127444=DIRECTION ( 'NONE',  ( -0.000000000000000000, -1.000000000000000000, -0.000000000000000000 ) ) ;
#127445=EDGE_CURVE ( 'NONE', #120897, #12970, #115729, .T. ) ;
#127446=DIRECTION ( 'NONE',  ( 0.000000000000000000, -0.000000000000000000, 1.000000000000000000 ) ) ;
#127447=ORIENTED_EDGE ( 'NONE', *, *, #64657, .F. ) ;
#127448=AXIS2_PLACEMENT_3D ( 'NONE', #14519, #61726, #81983 ) ;
#127449=DIRECTION ( 'NONE',  ( -0.000000000000000000, -1.000000000000000000, -0.000000000000000000 ) ) ;
#127450=DIRECTION ( 'NONE',  ( 0.000000000000000000, -0.9999939076577903929, 0.003490651415223739937 ) ) ;
#127451=DIRECTION ( 'NONE',  ( -0.000000000000000000, -1.000000000000000000, -0.000000000000000000 ) ) ;
#127452=DIRECTION ( 'NONE',  ( 0.000000000000000000, 0.000000000000000000, -1.000000000000000000 ) ) ;
#127453=LINE ( 'NONE', #77683, #18706 ) ;
#127454=ORIENTED_EDGE ( 'NONE', *, *, #94284, .F. ) ;
#127455=CARTESIAN_POINT ( 'NONE',  ( 11.69999999999990870, 2.500000000000000000, -4.430127018922202176 ) ) ;
#127456=DIRECTION ( 'NONE',  ( 0.000000000000000000, 0.000000000000000000, 1.000000000000000000 ) ) ;
#127457=CARTESIAN_POINT ( 'NONE',  ( -12.09999999999999432, 2.500000000000000000, 3.537306695894645081 ) ) ;
#127458=ORIENTED_EDGE ( 'NONE', *, *, #93307, .F. ) ;
#127460=VERTEX_POINT ( 'NONE', #128718 ) ;
#127461=ORIENTED_EDGE ( 'NONE', *, *, #80354, .T. ) ;
#127462=VERTEX_POINT ( 'NONE', #116270 ) ;
#127463=ORIENTED_EDGE ( 'NONE', *, *, #11842, .T. ) ;
#127464=DIRECTION ( 'NONE',  ( -4.274815082592931898E-19, -0.9999939076577903929, -0.003490651415223739937 ) ) ;
#127465=EDGE_CURVE ( 'NONE', #51670, #8233, #76031, .T. ) ;
#127466=ADVANCED_FACE ( 'NONE', ( #17415 ), #44644, .T. ) ;
#127467=CIRCLE ( 'NONE', #71037, 0.09999999999999982514 ) ;
#127468=CARTESIAN_POINT ( 'NONE',  ( -8.150000000000012790, 2.500000000000000000, 1.918653347947321564 ) ) ;
#127469=DIRECTION ( 'NONE',  ( 0.000000000000000000, 0.000000000000000000, -1.000000000000000000 ) ) ;
#127470=EDGE_CURVE ( 'NONE', #84006, #103567, #42604, .T. ) ;
#127471=DIRECTION ( 'NONE',  ( 0.000000000000000000, -0.9999939076577903929, 0.003490651415223739937 ) ) ;
#127472=ORIENTED_EDGE ( 'NONE', *, *, #72842, .T. ) ;
#127474=AXIS2_PLACEMENT_3D ( 'NONE', #113649, #74368, #102533 ) ;
#127475=DIRECTION ( 'NONE',  ( 0.000000000000000000, -0.000000000000000000, 1.000000000000000000 ) ) ;
#127476=ORIENTED_EDGE ( 'NONE', *, *, #96981, .F. ) ;
#127477=CARTESIAN_POINT ( 'NONE',  ( 24.00496409366837369, -0.9037364216029228903, -4.313973893095000456 ) ) ;
#127478=CARTESIAN_POINT ( 'NONE',  ( 15.40649769424532245, -2.500000000000000444, -5.817321162632588916 ) ) ;
#127479=AXIS2_PLACEMENT_3D ( 'NONE', #110772, #121250, #98369 ) ;
#127480=CARTESIAN_POINT ( 'NONE',  ( 9.599999999999914380, 12.50000000000000000, 5.022947341949748790 ) ) ;
#127481=PLANE ( 'NONE',  #96548 ) ;
#127482=EDGE_CURVE ( 'NONE', #14578, #72759, #122006, .T. ) ;
#127483=DIRECTION ( 'NONE',  ( -0.000000000000000000, 1.000000000000000000, -0.000000000000000000 ) ) ;
#127484=EDGE_CURVE ( 'NONE', #46669, #7958, #716, .T. ) ;
#127485=ORIENTED_EDGE ( 'NONE', *, *, #24710, .F. ) ;
#127486=AXIS2_PLACEMENT_3D ( 'NONE', #83344, #13930, #63699 ) ;
#127487=EDGE_CURVE ( 'NONE', #79310, #114635, #128038, .T. ) ;
#127488=EDGE_CURVE ( 'NONE', #93002, #78911, #68459, .T. ) ;
#127489=ORIENTED_EDGE ( 'NONE', *, *, #8794, .F. ) ;
#127490=ORIENTED_EDGE ( 'NONE', *, *, #16891, .T. ) ;
#127491=ORIENTED_EDGE ( 'NONE', *, *, #86209, .T. ) ;
#127492=CARTESIAN_POINT ( 'NONE',  ( -9.999999999999971578, 2.500000000000000000, -4.430127018922197735 ) ) ;
#127493=LINE ( 'NONE', #126844, #62420 ) ;
#127494=DIRECTION ( 'NONE',  ( 0.000000000000000000, 1.000000000000000000, 0.000000000000000000 ) ) ;
#127495=FACE_BOUND ( 'NONE', #1243, .T. ) ;
#127496=FACE_OUTER_BOUND ( 'NONE', #88548, .T. ) ;
#127497=CARTESIAN_POINT ( 'NONE',  ( 1.649999999999948841, 12.50000000000000000, 6.495190528383297135 ) ) ;
#127498=EDGE_CURVE ( 'NONE', #54010, #65711, #46796, .T. ) ;
#127499=CARTESIAN_POINT ( 'NONE',  ( -6.650000000000018119, 12.50000000000000000, -7.122917578226816815 ) ) ;
#127500=DIRECTION ( 'NONE',  ( -0.000000000000000000, -1.000000000000000000, -0.000000000000000000 ) ) ;
#127502=CARTESIAN_POINT ( 'NONE',  ( 6.849999999999927702, 2.500000000000000000, 2.511473670974873507 ) ) ;
#127503=DIRECTION ( 'NONE',  ( -0.000000000000000000, -1.000000000000000000, -0.000000000000000000 ) ) ;
#127504=CONICAL_SURFACE ( 'NONE', #20892, 0.09999999999999982514, 0.003490658503988666988 ) ;
#127505=VECTOR ( 'NONE', #29030, 1000.000000000000000 ) ;
#127506=CARTESIAN_POINT ( 'NONE',  ( 8.349999999999919709, 12.50000000000000000, 7.188010851410848723 ) ) ;
#127507=VERTEX_POINT ( 'NONE', #38390 ) ;
#127508=ORIENTED_EDGE ( 'NONE', *, *, #19719, .T. ) ;
#127509=VERTEX_POINT ( 'NONE', #107091 ) ;
#127510=ORIENTED_EDGE ( 'NONE', *, *, #100296, .T. ) ;
#127511=PLANE ( 'NONE',  #90406 ) ;
#127512=EDGE_CURVE ( 'NONE', #118058, #27024, #57364, .T. ) ;
#127513=FACE_BOUND ( 'NONE', #17762, .T. ) ;
#127514=CIRCLE ( 'NONE', #27158, 0.1000000000000000056 ) ;
#127516=ORIENTED_EDGE ( 'NONE', *, *, #79002, .F. ) ;
#127517=FACE_OUTER_BOUND ( 'NONE', #113012, .T. ) ;
#127518=DIRECTION ( 'NONE',  ( 0.000000000000000000, 0.000000000000000000, -1.000000000000000000 ) ) ;
#127519=DIRECTION ( 'NONE',  ( 0.000000000000000000, 1.000000000000000000, 0.000000000000000000 ) ) ;
#127520=AXIS2_PLACEMENT_3D ( 'NONE', #103197, #93383, #120899 ) ;
#127521=ORIENTED_EDGE ( 'NONE', *, *, #459, .F. ) ;
#127523=CARTESIAN_POINT ( 'NONE',  ( 19.01901804971389609, 2.576149587736915159, -2.431039412660902510 ) ) ;
#127524=AXIS2_PLACEMENT_3D ( 'NONE', #3360, #65492, #13807 ) ;
#127525=ADVANCED_FACE ( 'NONE', ( #56690 ), #80245, .T. ) ;
#127526=ORIENTED_EDGE ( 'NONE', *, *, #21939, .T. ) ;
#127527=CARTESIAN_POINT ( 'NONE',  ( -10.84999999999999964, 2.500000000000000000, 1.472243186433545459 ) ) ;
#127528=DIRECTION ( 'NONE',  ( 0.000000000000000000, 0.000000000000000000, -1.000000000000000000 ) ) ;
#127529=AXIS2_PLACEMENT_3D ( 'NONE', #117144, #55021, #27478 ) ;
#127530=VERTEX_POINT ( 'NONE', #7608 ) ;
#127531=DIRECTION ( 'NONE',  ( -0.000000000000000000, 1.000000000000000000, -0.000000000000000000 ) ) ;
#127532=CARTESIAN_POINT ( 'NONE',  ( 9.799999999999915445, 12.50000000000000000, -4.676537180435977881 ) ) ;
#127533=ORIENTED_EDGE ( 'NONE', *, *, #30711, .F. ) ;
#127534=CARTESIAN_POINT ( 'NONE',  ( -4.250072516143177381E-14, 2.500000000000000000, -3.637306695894650055 ) ) ;
#127535=AXIS2_PLACEMENT_3D ( 'NONE', #30770, #1918, #81145 ) ;
#127536=ORIENTED_EDGE ( 'NONE', *, *, #13783, .F. ) ;
#127537=EDGE_LOOP ( 'NONE', ( #108654, #104630, #8228, #126710 ) ) ;
#127538=EDGE_CURVE ( 'NONE', #26625, #18141, #73977, .T. ) ;
#127539=DIRECTION ( 'NONE',  ( -0.000000000000000000, -1.000000000000000000, -0.000000000000000000 ) ) ;
#127540=ORIENTED_EDGE ( 'NONE', *, *, #40950, .T. ) ;
#127541=DIRECTION ( 'NONE',  ( 0.000000000000000000, 1.000000000000000000, 0.000000000000000000 ) ) ;
#127542=FACE_BOUND ( 'NONE', #65395, .T. ) ;
#127543=ORIENTED_EDGE ( 'NONE', *, *, #55468, .F. ) ;
#127545=ORIENTED_EDGE ( 'NONE', *, *, #54881, .F. ) ;
#127547=DIRECTION ( 'NONE',  ( 0.000000000000000000, 0.000000000000000000, 1.000000000000000000 ) ) ;
#127548=DIRECTION ( 'NONE',  ( 0.000000000000000000, 0.000000000000000000, 1.000000000000000000 ) ) ;
#127549=DIRECTION ( 'NONE',  ( 0.000000000000000000, 1.000000000000000000, 0.000000000000000000 ) ) ;
#127550=CARTESIAN_POINT ( 'NONE',  ( -5.400000000000023448, 12.50000000000000000, -4.957854068765716882 ) ) ;
#127551=ORIENTED_EDGE ( 'NONE', *, *, #96124, .F. ) ;
#127552=VERTEX_POINT ( 'NONE', #29213 ) ;
#127553=CARTESIAN_POINT ( 'NONE',  ( 1.049999999999954081, 2.500000000000000000, -6.148780366869526226 ) ) ;
#127554=CARTESIAN_POINT ( 'NONE',  ( 16.86635082839108080, -0.4716143926291173072, 5.778906370536277315 ) ) ;
#127555=AXIS2_PLACEMENT_3D ( 'NONE', #47566, #117551, #116921 ) ;
#127556=CARTESIAN_POINT ( 'NONE',  ( 7.949999999999922018, 12.50000000000000000, 6.560283801567334372 ) ) ;
#127557=VERTEX_POINT ( 'NONE', #126759 ) ;
#127558=VERTEX_POINT ( 'NONE', #26614 ) ;
#127559=EDGE_LOOP ( 'NONE', ( #49663, #86155, #24110, #54367 ) ) ;
#127560=CONICAL_SURFACE ( 'NONE', #41891, 0.09999999999999982514, 0.003490658503988666988 ) ;
#127561=CARTESIAN_POINT ( 'NONE',  ( 13.94999999999989448, 2.500000000000000000, -2.411473670974877859 ) ) ;
#127562=CARTESIAN_POINT ( 'NONE',  ( -4.150000000000024336, 2.500000000000000000, -2.857883832488653741 ) ) ;
#127563=EDGE_CURVE ( 'NONE', #97855, #107047, #7053, .T. ) ;
#127564=AXIS2_PLACEMENT_3D ( 'NONE', #19927, #120694, #71593 ) ;
#127565=AXIS2_PLACEMENT_3D ( 'NONE', #72923, #113483, #23167 ) ;
#127566=CARTESIAN_POINT ( 'NONE',  ( -9.400000000000009237, 2.500000000000000000, -4.083716857408422385 ) ) ;
#127567=DIRECTION ( 'NONE',  ( 0.000000000000000000, 0.000000000000000000, 1.000000000000000000 ) ) ;
#127568=DIRECTION ( 'NONE',  ( -0.000000000000000000, -1.000000000000000000, -0.000000000000000000 ) ) ;
#127569=CARTESIAN_POINT ( 'NONE',  ( 6.249999999999932498, 2.500000000000000000, -5.802370205355749988 ) ) ;
#127570=CARTESIAN_POINT ( 'NONE',  ( 2.699999999999944666, 2.500000000000000000, 4.676537180435972552 ) ) ;
#127572=ADVANCED_FACE ( 'NONE', ( #69108 ), #804, .T. ) ;
#127573=ORIENTED_EDGE ( 'NONE', *, *, #115858, .T. ) ;
#127574=VERTEX_POINT ( 'NONE', #47553 ) ;
#127575=FACE_OUTER_BOUND ( 'NONE', #7904, .T. ) ;
#127577=ADVANCED_FACE ( 'NONE', ( #37729 ), #77631, .T. ) ;
#127578=ORIENTED_EDGE ( 'NONE', *, *, #49029, .T. ) ;
#127579=EDGE_CURVE ( 'NONE', #53467, #25412, #9130, .T. ) ;
#127580=ORIENTED_EDGE ( 'NONE', *, *, #4481, .T. ) ;
#127581=EDGE_CURVE ( 'NONE', #67817, #71756, #98549, .T. ) ;
#127583=DIRECTION ( 'NONE',  ( 0.000000000000000000, -0.9999939076577903929, 0.003490651415223739937 ) ) ;
#127584=ADVANCED_FACE ( 'NONE', ( #20670 ), #111633, .T. ) ;
#127585=DIRECTION ( 'NONE',  ( 0.000000000000000000, -0.9999939076577903929, 0.003490651415223739937 ) ) ;
#127586=DIRECTION ( 'NONE',  ( 0.000000000000000000, 0.000000000000000000, -1.000000000000000000 ) ) ;
#127587=LINE ( 'NONE', #37911, #109221 ) ;
#127588=DIRECTION ( 'NONE',  ( 0.000000000000000000, 0.000000000000000000, 1.000000000000000000 ) ) ;
#127589=LINE ( 'NONE', #68663, #84480 ) ;
#127590=ORIENTED_EDGE ( 'NONE', *, *, #39093, .F. ) ;
#127591=CARTESIAN_POINT ( 'NONE',  ( -9.150000000000009237, 2.500000000000000000, -6.395190528383296602 ) ) ;
#127592=EDGE_CURVE ( 'NONE', #12208, #21305, #113781, .T. ) ;
#127593=CARTESIAN_POINT ( 'NONE',  ( 11.44999999999990514, 12.50000000000000000, -6.148780366869526226 ) ) ;
#127594=EDGE_CURVE ( 'NONE', #105260, #98489, #117875, .T. ) ;
#127596=EDGE_CURVE ( 'NONE', #76681, #3042, #121428, .T. ) ;
#127597=AXIS2_PLACEMENT_3D ( 'NONE', #73161, #74449, #112450 ) ;
#127598=VERTEX_POINT ( 'NONE', #109695 ) ;
#127599=ORIENTED_EDGE ( 'NONE', *, *, #38193, .F. ) ;
#127600=ORIENTED_EDGE ( 'NONE', *, *, #38427, .F. ) ;
#127601=ORIENTED_EDGE ( 'NONE', *, *, #120188, .T. ) ;
#127602=DIRECTION ( 'NONE',  ( 0.000000000000000000, 0.000000000000000000, -1.000000000000000000 ) ) ;
#127603=DIRECTION ( 'NONE',  ( 0.000000000000000000, 1.000000000000000000, 0.000000000000000000 ) ) ;
#127604=VECTOR ( 'NONE', #52935, 1000.000000000000000 ) ;
#127605=ORIENTED_EDGE ( 'NONE', *, *, #92829, .T. ) ;
#127606=DIRECTION ( 'NONE',  ( -0.000000000000000000, -1.000000000000000000, -0.000000000000000000 ) ) ;
#127607=CARTESIAN_POINT ( 'NONE',  ( 2.500000000000002220, -0.9166666666666694052, -9.999999999999998224 ) ) ;
#127608=DIRECTION ( 'NONE',  ( 0.000000000000000000, 0.000000000000000000, 1.000000000000000000 ) ) ;
#127609=CARTESIAN_POINT ( 'NONE',  ( -14.54999999999998472, 12.50000000000000000, -2.099970236277062252 ) ) ;
#127610=ORIENTED_EDGE ( 'NONE', *, *, #127433, .F. ) ;
#127611=DIRECTION ( 'NONE',  ( 0.000000000000000000, -0.9999939076577903929, 0.003490651415223739937 ) ) ;
#127612=DIRECTION ( 'NONE',  ( 0.000000000000000000, 0.000000000000000000, -1.000000000000000000 ) ) ;
#127613=ORIENTED_EDGE ( 'NONE', *, *, #127066, .F. ) ;
#127614=AXIS2_PLACEMENT_3D ( 'NONE', #68867, #43153, #69503 ) ;
#127615=ORIENTED_EDGE ( 'NONE', *, *, #7997, .F. ) ;
#127616=ORIENTED_EDGE ( 'NONE', *, *, #107949, .T. ) ;
#127617=DIRECTION ( 'NONE',  ( 0.000000000000000000, 1.000000000000000000, 0.000000000000000000 ) ) ;
#127618=AXIS2_PLACEMENT_3D ( 'NONE', #118452, #8487, #38639 ) ;
#127619=DIRECTION ( 'NONE',  ( 0.000000000000000000, 1.000000000000000000, 0.000000000000000000 ) ) ;
#127620=CIRCLE ( 'NONE', #89961, 0.1000000000000002554 ) ;
#127621=ORIENTED_EDGE ( 'NONE', *, *, #104778, .T. ) ;
#127622=FACE_OUTER_BOUND ( 'NONE', #46799, .T. ) ;
#127623=DIRECTION ( 'NONE',  ( -0.000000000000000000, -1.000000000000000000, -0.000000000000000000 ) ) ;
#127624=FACE_OUTER_BOUND ( 'NONE', #111526, .T. ) ;
#127626=ADVANCED_FACE ( 'NONE', ( #119495 ), #84441, .T. ) ;
#127627=EDGE_CURVE ( 'NONE', #26903, #110184, #69760, .T. ) ;
#127628=VERTEX_POINT ( 'NONE', #100501 ) ;
#127629=DIRECTION ( 'NONE',  ( -0.000000000000000000, 1.000000000000000000, -0.000000000000000000 ) ) ;
#127630=ADVANCED_FACE ( 'NONE', ( #40971 ), #44739, .T. ) ;
#127631=ORIENTED_EDGE ( 'NONE', *, *, #64795, .T. ) ;
#127632=ORIENTED_EDGE ( 'NONE', *, *, #76212, .T. ) ;
#127633=DIRECTION ( 'NONE',  ( 0.000000000000000000, 0.000000000000000000, 1.000000000000000000 ) ) ;
#127634=FACE_OUTER_BOUND ( 'NONE', #9636, .T. ) ;
#127635=FACE_BOUND ( 'NONE', #62890, .T. ) ;
#127636=CARTESIAN_POINT ( 'NONE',  ( -13.74999999999998757, 12.50000000000000000, -2.857883832488651521 ) ) ;
#127637=PLANE ( 'NONE',  #123852 ) ;
#127638=EDGE_CURVE ( 'NONE', #66996, #27297, #120790, .T. ) ;
#127639=DIRECTION ( 'NONE',  ( 0.000000000000000000, 0.000000000000000000, -1.000000000000000000 ) ) ;
#127640=VECTOR ( 'NONE', #54003, 1000.000000000000000 ) ;
#127641=CONICAL_SURFACE ( 'NONE', #94192, 0.1000000000000002554, 0.003490658503988666988 ) ;
#127642=ORIENTED_EDGE ( 'NONE', *, *, #45471, .F. ) ;
#127643=CARTESIAN_POINT ( 'NONE',  ( -9.350000000000006750, 2.500000000000000000, -2.511473670974877948 ) ) ;
#127644=CIRCLE ( 'NONE', #92133, 0.06509327318403745899 ) ;
#127645=DIRECTION ( 'NONE',  ( -4.274815082592931898E-19, -0.9999939076577903929, -0.003490651415223739937 ) ) ;
#127646=FACE_OUTER_BOUND ( 'NONE', #30726, .T. ) ;
#127647=DIRECTION ( 'NONE',  ( -0.000000000000000000, 1.000000000000000000, -0.000000000000000000 ) ) ;
#127648=ORIENTED_EDGE ( 'NONE', *, *, #107484, .T. ) ;
#127649=DIRECTION ( 'NONE',  ( 0.000000000000000000, 0.000000000000000000, 1.000000000000000000 ) ) ;
#127650=CONICAL_SURFACE ( 'NONE', #81680, 0.1000000000000002554, 0.003490658503988666988 ) ;
#127651=DIRECTION ( 'NONE',  ( 0.000000000000000000, 0.000000000000000000, 1.000000000000000000 ) ) ;
#127652=ORIENTED_EDGE ( 'NONE', *, *, #83984, .T. ) ;
#127653=ORIENTED_EDGE ( 'NONE', *, *, #110806, .F. ) ;
#127654=DIRECTION ( 'NONE',  ( -4.274815082592931898E-19, -0.9999939076577903929, -0.003490651415223739937 ) ) ;
#127655=CARTESIAN_POINT ( 'NONE',  ( 9.999999999999948486, 12.50000000000000000, -4.330127018922201643 ) ) ;
#127656=ADVANCED_FACE ( 'NONE', ( #21295 ), #120153, .T. ) ;
#127657=FACE_BOUND ( 'NONE', #20865, .T. ) ;
#127658=CARTESIAN_POINT ( 'NONE',  ( 4.999999999999935163, 2.500000000000000000, 3.637306695894644726 ) ) ;
#127659=EDGE_LOOP ( 'NONE', ( #72131, #74081, #86424, #9350 ) ) ;
#127660=DIRECTION ( 'NONE',  ( 0.000000000000000000, -0.9999939076577903929, 0.003490651415223739937 ) ) ;
#127661=EDGE_LOOP ( 'NONE', ( #61212, #50856, #82422, #6188 ) ) ;
#127662=VERTEX_POINT ( 'NONE', #30507 ) ;
#127663=DIRECTION ( 'NONE',  ( -0.000000000000000000, -1.000000000000000000, -0.000000000000000000 ) ) ;
#127665=ORIENTED_EDGE ( 'NONE', *, *, #53007, .F. ) ;
#127666=DIRECTION ( 'NONE',  ( -0.000000000000000000, -1.000000000000000000, -0.000000000000000000 ) ) ;
#127667=DIRECTION ( 'NONE',  ( -0.000000000000000000, 1.000000000000000000, -0.000000000000000000 ) ) ;
#127668=EDGE_CURVE ( 'NONE', #50344, #57584, #110330, .T. ) ;
#127669=FACE_OUTER_BOUND ( 'NONE', #66797, .T. ) ;
#127670=LINE ( 'NONE', #119145, #11266 ) ;
#127671=CIRCLE ( 'NONE', #18909, 0.1000000000000000472 ) ;
#127672=EDGE_CURVE ( 'NONE', #62361, #1969, #61473, .T. ) ;
#127673=CIRCLE ( 'NONE', #123555, 0.09999999999999982514 ) ;
#127674=ORIENTED_EDGE ( 'NONE', *, *, #53101, .T. ) ;
#127675=DIRECTION ( 'NONE',  ( 0.000000000000000000, 1.000000000000000000, 0.000000000000000000 ) ) ;
#127676=DIRECTION ( 'NONE',  ( 0.000000000000000000, 1.000000000000000000, 0.000000000000000000 ) ) ;
#127677=CARTESIAN_POINT ( 'NONE',  ( -5.600000000000023626, 12.50000000000000000, -4.676537180435977881 ) ) ;
#127678=CARTESIAN_POINT ( 'NONE',  ( -6.250000000000019540, 2.500000000000000000, -2.757883832488654097 ) ) ;
#127680=DIRECTION ( 'NONE',  ( 0.000000000000000000, 0.000000000000000000, 1.000000000000000000 ) ) ;
#127681=EDGE_LOOP ( 'NONE', ( #24638, #96004, #62339, #115991 ) ) ;
#127682=EDGE_CURVE ( 'NONE', #59852, #37316, #32230, .T. ) ;
#127683=DIRECTION ( 'NONE',  ( -0.000000000000000000, 1.000000000000000000, -0.000000000000000000 ) ) ;
#127684=CIRCLE ( 'NONE', #100497, 0.09999999999999982514 ) ;
#127685=VERTEX_POINT ( 'NONE', #89175 ) ;
#127686=CARTESIAN_POINT ( 'NONE',  ( -10.65000000000000391, 2.500000000000000000, -6.148780366869522673 ) ) ;
#127687=CIRCLE ( 'NONE', #58743, 0.06509327318403745899 ) ;
#127688=DIRECTION ( 'NONE',  ( 0.000000000000000000, 0.000000000000000000, -1.000000000000000000 ) ) ;
#127690=LINE ( 'NONE', #68118, #36131 ) ;
#127691=ORIENTED_EDGE ( 'NONE', *, *, #33778, .F. ) ;
#127692=DIRECTION ( 'NONE',  ( 0.000000000000000000, 0.000000000000000000, 1.000000000000000000 ) ) ;
#127693=CARTESIAN_POINT ( 'NONE',  ( 1.249999999999953815, 2.500000000000000000, -2.857883832488653741 ) ) ;
#127694=EDGE_CURVE ( 'NONE', #58594, #91328, #59425, .T. ) ;
#127695=FACE_OUTER_BOUND ( 'NONE', #13363, .T. ) ;
#127696=DIRECTION ( 'NONE',  ( 0.000000000000000000, 0.000000000000000000, 1.000000000000000000 ) ) ;
#127697=DIRECTION ( 'NONE',  ( -4.274815082592931898E-19, -0.9999939076577903929, -0.003490651415223739937 ) ) ;
#127698=CIRCLE ( 'NONE', #85830, 0.06509327318403745899 ) ;
#127699=ORIENTED_EDGE ( 'NONE', *, *, #103376, .F. ) ;
#127700=ORIENTED_EDGE ( 'NONE', *, *, #16430, .F. ) ;
#127701=CARTESIAN_POINT ( 'NONE',  ( 2.899999999999946620, 2.500000000000000000, -3.637306695894650055 ) ) ;
#127702=ORIENTED_EDGE ( 'NONE', *, *, #36732, .F. ) ;
#127703=CARTESIAN_POINT ( 'NONE',  ( 1.249999999999952038, 2.500000000000000000, 2.857883832488649301 ) ) ;
#127704=EDGE_LOOP ( 'NONE', ( #100994, #14909 ) ) ;
#127705=ORIENTED_EDGE ( 'NONE', *, *, #72342, .T. ) ;
#127706=ORIENTED_EDGE ( 'NONE', *, *, #92685, .T. ) ;
#127707=DIRECTION ( 'NONE',  ( 0.000000000000000000, 1.000000000000000000, 0.000000000000000000 ) ) ;
#127708=AXIS2_PLACEMENT_3D ( 'NONE', #103346, #82427, #83700 ) ;
#127709=CARTESIAN_POINT ( 'NONE',  ( 11.64999999999990443, 2.500000000000000000, 2.957883832488649389 ) ) ;
#127710=DIRECTION ( 'NONE',  ( -4.274815082592931898E-19, -0.9999939076577903929, -0.003490651415223739937 ) ) ;
#127711=EDGE_CURVE ( 'NONE', #27444, #2801, #86574, .T. ) ;
#127712=DIRECTION ( 'NONE',  ( -0.000000000000000000, -1.000000000000000000, -0.000000000000000000 ) ) ;
#127713=AXIS2_PLACEMENT_3D ( 'NONE', #103694, #23843, #2241 ) ;
#127714=CARTESIAN_POINT ( 'NONE',  ( -4.150000000000025224, 2.500000000000000000, -1.372243186433550033 ) ) ;
#127715=FACE_OUTER_BOUND ( 'NONE', #52683, .T. ) ;
#127716=CARTESIAN_POINT ( 'NONE',  ( -5.800000000000018474, 2.500000000000000000, 4.230127018922196669 ) ) ;
#127717=CARTESIAN_POINT ( 'NONE',  ( -9.150000000000011013, 12.50000000000000000, -5.802370205355744659 ) ) ;
#127718=ORIENTED_EDGE ( 'NONE', *, *, #65031, .T. ) ;
#127719=EDGE_CURVE ( 'NONE', #31303, #7039, #30169, .T. ) ;
#127720=ORIENTED_EDGE ( 'NONE', *, *, #82875, .F. ) ;
#127721=VERTEX_POINT ( 'NONE', #98335 ) ;
#127722=EDGE_LOOP ( 'NONE', ( #39019, #86454, #92491, #47221 ) ) ;
#127723=LINE ( 'NONE', #106159, #27717 ) ;
#127724=EDGE_CURVE ( 'NONE', #101537, #73886, #117306, .T. ) ;
#127725=EDGE_LOOP ( 'NONE', ( #108322, #119070, #96467, #27206 ) ) ;
#127726=ADVANCED_FACE ( 'NONE', ( #27037 ), #17619, .T. ) ;
#127727=ORIENTED_EDGE ( 'NONE', *, *, #73753, .T. ) ;
#127728=EDGE_CURVE ( 'NONE', #73897, #39360, #127807, .T. ) ;
#127729=EDGE_CURVE ( 'NONE', #67328, #36126, #38144, .T. ) ;
#127730=PLANE ( 'NONE',  #74887 ) ;
#127731=CARTESIAN_POINT ( 'NONE',  ( -7.500000000000011546, 2.500000000000000000, 3.737306695894644371 ) ) ;
#127732=CARTESIAN_POINT ( 'NONE',  ( -4.350000000000027178, 2.500000000000000000, -6.148780366869526226 ) ) ;
#127733=DIRECTION ( 'NONE',  ( -0.000000000000000000, -1.000000000000000000, -0.000000000000000000 ) ) ;
#127734=ADVANCED_FACE ( 'NONE', ( #129126 ), #94905, .T. ) ;
#127735=CIRCLE ( 'NONE', #62987, 0.06509327318403745899 ) ;
#127736=DIRECTION ( 'NONE',  ( -0.000000000000000000, -1.000000000000000000, -0.000000000000000000 ) ) ;
#127738=CONICAL_SURFACE ( 'NONE', #29544, 0.1000000000000000472, 0.003490658503988666988 ) ;
#127739=CIRCLE ( 'NONE', #121467, 0.09999999999999982514 ) ;
#127740=EDGE_CURVE ( 'NONE', #103358, #1125, #103315, .T. ) ;
#127741=EDGE_CURVE ( 'NONE', #117845, #51418, #19694, .T. ) ;
#127742=DIRECTION ( 'NONE',  ( -0.000000000000000000, 1.000000000000000000, -0.000000000000000000 ) ) ;
#127743=EDGE_CURVE ( 'NONE', #95554, #55527, #109580, .T. ) ;
#127744=ORIENTED_EDGE ( 'NONE', *, *, #120851, .T. ) ;
#127745=DIRECTION ( 'NONE',  ( 0.000000000000000000, 0.000000000000000000, -1.000000000000000000 ) ) ;
#127746=CONICAL_SURFACE ( 'NONE', #71299, 0.1000000000000000472, 0.003490658503988666988 ) ;
#127747=ADVANCED_FACE ( 'NONE', ( #106862 ), #49270, .T. ) ;
#127748=EDGE_LOOP ( 'NONE', ( #102747, #3779 ) ) ;
#127749=CARTESIAN_POINT ( 'NONE',  ( 3.349999999999945466, 2.500000000000000000, -6.595190528383302109 ) ) ;
#127750=ORIENTED_EDGE ( 'NONE', *, *, #113217, .T. ) ;
#127751=AXIS2_PLACEMENT_3D ( 'NONE', #62535, #91334, #71056 ) ;
#127752=ORIENTED_EDGE ( 'NONE', *, *, #67135, .T. ) ;
#127753=EDGE_CURVE ( 'NONE', #104203, #35289, #51007, .T. ) ;
#127754=DIRECTION ( 'NONE',  ( 0.000000000000000000, 1.000000000000000000, 0.000000000000000000 ) ) ;
#127755=DIRECTION ( 'NONE',  ( 0.000000000000000000, -0.9999939076577903929, 0.003490651415223739937 ) ) ;
#127756=DIRECTION ( 'NONE',  ( 0.000000000000000000, -0.000000000000000000, 1.000000000000000000 ) ) ;
#127757=CARTESIAN_POINT ( 'NONE',  ( -10.84999999999999964, 2.500000000000000000, 7.288010851410849256 ) ) ;
#127759=ORIENTED_EDGE ( 'NONE', *, *, #61935, .T. ) ;
#127760=DIRECTION ( 'NONE',  ( 0.000000000000000000, 0.000000000000000000, 1.000000000000000000 ) ) ;
#127761=DIRECTION ( 'NONE',  ( 0.000000000000000000, 0.000000000000000000, -1.000000000000000000 ) ) ;
#127762=CARTESIAN_POINT ( 'NONE',  ( 3.099999999999945022, 2.500000000000000000, -4.576537180435978236 ) ) ;
#127763=DIRECTION ( 'NONE',  ( 0.000000000000000000, 0.000000000000000000, 1.000000000000000000 ) ) ;
#127764=DIRECTION ( 'NONE',  ( 0.000000000000000000, -0.000000000000000000, 1.000000000000000000 ) ) ;
#127765=ORIENTED_EDGE ( 'NONE', *, *, #45852, .T. ) ;
#127766=VECTOR ( 'NONE', #26767, 1000.000000000000000 ) ;
#127767=ORIENTED_EDGE ( 'NONE', *, *, #56068, .F. ) ;
#127768=CARTESIAN_POINT ( 'NONE',  ( -8.350000000000008527, 2.500000000000000000, 5.802370205355744659 ) ) ;
#127769=ORIENTED_EDGE ( 'NONE', *, *, #17340, .F. ) ;
#127770=DIRECTION ( 'NONE',  ( 0.000000000000000000, 0.000000000000000000, 1.000000000000000000 ) ) ;
#127771=CONICAL_SURFACE ( 'NONE', #102630, 0.1000000000000000472, 0.003490658503988666988 ) ;
#127772=DIRECTION ( 'NONE',  ( 0.000000000000000000, -0.9999939076577903929, 0.003490651415223739937 ) ) ;
#127773=AXIS2_PLACEMENT_3D ( 'NONE', #36952, #25836, #76872 ) ;
#127774=EDGE_LOOP ( 'NONE', ( #120859, #71706 ) ) ;
#127776=CARTESIAN_POINT ( 'NONE',  ( 6.249999999999934275, 12.50000000000000000, -7.188010851410854052 ) ) ;
#127778=CARTESIAN_POINT ( 'NONE',  ( 12.04999999999990834, 12.50000000000000000, -2.165063509461101710 ) ) ;
#127779=EDGE_LOOP ( 'NONE', ( #91810, #70540, #50507, #15305 ) ) ;
#127780=VECTOR ( 'NONE', #123439, 1000.000000000000000 ) ;
#127781=VECTOR ( 'NONE', #87006, 1000.000000000000000 ) ;
#127782=EDGE_CURVE ( 'NONE', #70962, #111188, #77420, .T. ) ;
#127783=CARTESIAN_POINT ( 'NONE',  ( 13.09999999999989839, 2.500000000000000000, -0.4464101615137783252 ) ) ;
#127784=FACE_OUTER_BOUND ( 'NONE', #105913, .T. ) ;
#127785=EDGE_CURVE ( 'NONE', #33867, #73941, #128379, .T. ) ;
#127786=ORIENTED_EDGE ( 'NONE', *, *, #78420, .F. ) ;
#127787=DIRECTION ( 'NONE',  ( -0.000000000000000000, -1.000000000000000000, -0.000000000000000000 ) ) ;
#127788=DIRECTION ( 'NONE',  ( 0.000000000000000000, -0.9999939076577903929, 0.003490651415223739937 ) ) ;
#127789=FACE_OUTER_BOUND ( 'NONE', #96554, .T. ) ;
#127790=CIRCLE ( 'NONE', #98524, 0.1000000000000000472 ) ;
#127791=ADVANCED_FACE ( 'NONE', ( #57790 ), #92859, .T. ) ;
#127792=CONICAL_SURFACE ( 'NONE', #117291, 0.09999999999999999167, 0.003490658503988666988 ) ;
#127793=ORIENTED_EDGE ( 'NONE', *, *, #30858, .F. ) ;
#127794=FACE_OUTER_BOUND ( 'NONE', #66614, .T. ) ;
#127795=AXIS2_PLACEMENT_3D ( 'NONE', #22028, #101858, #112327 ) ;
#127796=VERTEX_POINT ( 'NONE', #108158 ) ;
#127797=CARTESIAN_POINT ( 'NONE',  ( -12.89999999999999147, 2.500000000000000000, -5.022947341949751454 ) ) ;
#127798=DIRECTION ( 'NONE',  ( 0.000000000000000000, 0.000000000000000000, 1.000000000000000000 ) ) ;
#127799=AXIS2_PLACEMENT_3D ( 'NONE', #124750, #84169, #124100 ) ;
#127800=LINE ( 'NONE', #47966, #16197 ) ;
#127801=ORIENTED_EDGE ( 'NONE', *, *, #84589, .T. ) ;
#127802=DIRECTION ( 'NONE',  ( 0.000000000000000000, 0.000000000000000000, 1.000000000000000000 ) ) ;
#127803=DIRECTION ( 'NONE',  ( 0.000000000000000000, 0.000000000000000000, -1.000000000000000000 ) ) ;
#127804=CIRCLE ( 'NONE', #52588, 0.1000000000000002554 ) ;
#127805=CIRCLE ( 'NONE', #102665, 0.09999999999999982514 ) ;
#127806=ORIENTED_EDGE ( 'NONE', *, *, #72490, .T. ) ;
#127807=LINE ( 'NONE', #130, #78192 ) ;
#127808=ORIENTED_EDGE ( 'NONE', *, *, #9680, .F. ) ;
#127809=DIRECTION ( 'NONE',  ( -0.000000000000000000, -1.000000000000000000, -0.000000000000000000 ) ) ;
#127810=EDGE_LOOP ( 'NONE', ( #40797, #120461 ) ) ;
#127811=LINE ( 'NONE', #97065, #117392 ) ;
#127812=LINE ( 'NONE', #8030, #58399 ) ;
#127813=ORIENTED_EDGE ( 'NONE', *, *, #110002, .T. ) ;
#127814=EDGE_LOOP ( 'NONE', ( #107072, #127691, #35231, #121033 ) ) ;
#127815=DIRECTION ( 'NONE',  ( 0.000000000000000000, 1.000000000000000000, 0.000000000000000000 ) ) ;
#127816=CARTESIAN_POINT ( 'NONE',  ( 12.89999999999989910, 12.50000000000000000, -0.6928203230275542523 ) ) ;
#127817=VERTEX_POINT ( 'NONE', #18495 ) ;
#127818=FACE_OUTER_BOUND ( 'NONE', #126247, .T. ) ;
#127819=EDGE_CURVE ( 'NONE', #116265, #34015, #48946, .T. ) ;
#127820=DIRECTION ( 'NONE',  ( -0.000000000000000000, -1.000000000000000000, -0.000000000000000000 ) ) ;
#127821=AXIS2_PLACEMENT_3D ( 'NONE', #7207, #89018, #47159 ) ;
#127822=CARTESIAN_POINT ( 'NONE',  ( -10.20000000000000284, 12.50000000000000000, 3.983716857408420964 ) ) ;
#127823=DIRECTION ( 'NONE',  ( 0.000000000000000000, 1.000000000000000000, 0.000000000000000000 ) ) ;
#127824=AXIS2_PLACEMENT_3D ( 'NONE', #65926, #6987, #27287 ) ;
#127825=AXIS2_PLACEMENT_3D ( 'NONE', #51293, #61753, #110820 ) ;
#127826=DIRECTION ( 'NONE',  ( -0.000000000000000000, 1.000000000000000000, -0.000000000000000000 ) ) ;
#127827=ADVANCED_FACE ( 'NONE', ( #98993 ), #115828, .T. ) ;
#127828=DIRECTION ( 'NONE',  ( -0.000000000000000000, 1.000000000000000000, -0.000000000000000000 ) ) ;
#127829=AXIS2_PLACEMENT_3D ( 'NONE', #100730, #28793, #58256 ) ;
#127830=ORIENTED_EDGE ( 'NONE', *, *, #116951, .T. ) ;
#127831=AXIS2_PLACEMENT_3D ( 'NONE', #24678, #46241, #14189 ) ;
#127832=ORIENTED_EDGE ( 'NONE', *, *, #32013, .F. ) ;
#127833=VERTEX_POINT ( 'NONE', #60384 ) ;
#127834=VERTEX_POINT ( 'NONE', #120568 ) ;
#127835=DIRECTION ( 'NONE',  ( -0.000000000000000000, 1.000000000000000000, -0.000000000000000000 ) ) ;
#127836=CARTESIAN_POINT ( 'NONE',  ( 3.349999999999941025, 12.50000000000000000, 7.253104124594885960 ) ) ;
#127837=AXIS2_PLACEMENT_3D ( 'NONE', #117387, #38897, #67663 ) ;
#127838=ADVANCED_FACE ( 'NONE', ( #31547 ), #99119, .T. ) ;
#127839=PLANE ( 'NONE',  #78194 ) ;
#127840=VERTEX_POINT ( 'NONE', #782 ) ;
#127841=FACE_BOUND ( 'NONE', #78, .T. ) ;
#127842=ORIENTED_EDGE ( 'NONE', *, *, #71686, .T. ) ;
#127843=CARTESIAN_POINT ( 'NONE',  ( -4.550000000000022915, 2.500000000000000000, 2.165063509461097713 ) ) ;
#127844=PLANE ( 'NONE',  #54320 ) ;
#127845=PLANE ( 'NONE',  #93177 ) ;
#127846=DIRECTION ( 'NONE',  ( 0.000000000000000000, 0.000000000000000000, -1.000000000000000000 ) ) ;
#127848=CARTESIAN_POINT ( 'NONE',  ( -9.400000000000007461, 2.500000000000000000, -0.2464101615137783419 ) ) ;
#127849=CARTESIAN_POINT ( 'NONE',  ( 3.749999999999978684, 12.50000000000000000, -6.495190528383302464 ) ) ;
#127850=DIRECTION ( 'NONE',  ( -0.000000000000000000, -1.000000000000000000, -0.000000000000000000 ) ) ;
#127851=EDGE_CURVE ( 'NONE', #114403, #93012, #110737, .T. ) ;
#127852=FACE_OUTER_BOUND ( 'NONE', #122107, .T. ) ;
#127853=FACE_OUTER_BOUND ( 'NONE', #64178, .T. ) ;
#127854=ORIENTED_EDGE ( 'NONE', *, *, #96867, .T. ) ;
#127855=ORIENTED_EDGE ( 'NONE', *, *, #174, .T. ) ;
#127856=ORIENTED_EDGE ( 'NONE', *, *, #53653, .T. ) ;
#127857=ORIENTED_EDGE ( 'NONE', *, *, #47323, .T. ) ;
#127858=CARTESIAN_POINT ( 'NONE',  ( -12.09999999999999432, 2.500000000000000000, 4.922947341949748257 ) ) ;
#127859=FACE_OUTER_BOUND ( 'NONE', #114825, .T. ) ;
#127860=ORIENTED_EDGE ( 'NONE', *, *, #33005, .T. ) ;
#127861=ORIENTED_EDGE ( 'NONE', *, *, #108026, .F. ) ;
#127862=ORIENTED_EDGE ( 'NONE', *, *, #87524, .F. ) ;
#127863=LINE ( 'NONE', #6773, #119042 ) ;
#127864=AXIS2_PLACEMENT_3D ( 'NONE', #122942, #65286, #114394 ) ;
#127865=CIRCLE ( 'NONE', #56822, 0.06509327318403745899 ) ;
#127866=CARTESIAN_POINT ( 'NONE',  ( -10.85000000000000142, 2.500000000000000000, -2.857883832488649745 ) ) ;
#127867=DIRECTION ( 'NONE',  ( 0.000000000000000000, 0.000000000000000000, 1.000000000000000000 ) ) ;
#127868=CARTESIAN_POINT ( 'NONE',  ( 11.64999999999990798, 2.500000000000000000, 7.188010851410848723 ) ) ;
#127869=DIRECTION ( 'NONE',  ( -0.000000000000000000, 1.000000000000000000, -0.000000000000000000 ) ) ;
#127870=DIRECTION ( 'NONE',  ( 0.000000000000000000, 0.000000000000000000, 1.000000000000000000 ) ) ;
#127872=VERTEX_POINT ( 'NONE', #72121 ) ;
#127873=AXIS2_PLACEMENT_3D ( 'NONE', #56925, #7192, #55011 ) ;
#127874=FACE_OUTER_BOUND ( 'NONE', #20495, .T. ) ;
#127875=ORIENTED_EDGE ( 'NONE', *, *, #74047, .T. ) ;
#127876=AXIS2_PLACEMENT_3D ( 'NONE', #122608, #23109, #1526 ) ;
#127877=ADVANCED_FACE ( 'NONE', ( #62306 ), #40744, .T. ) ;
#127878=ORIENTED_EDGE ( 'NONE', *, *, #76474, .T. ) ;
#127879=AXIS2_PLACEMENT_3D ( 'NONE', #39086, #98599, #76414 ) ;
#127880=ORIENTED_EDGE ( 'NONE', *, *, #1382, .T. ) ;
#127881=AXIS2_PLACEMENT_3D ( 'NONE', #80043, #81968, #121899 ) ;
#127882=CARTESIAN_POINT ( 'NONE',  ( 10.64999999999990976, 12.50000000000000000, -6.841600689897077814 ) ) ;
#127883=ORIENTED_EDGE ( 'NONE', *, *, #37139, .T. ) ;
#127884=EDGE_CURVE ( 'NONE', #27857, #378, #82589, .T. ) ;
#127885=ORIENTED_EDGE ( 'NONE', *, *, #61977, .F. ) ;
#127886=EDGE_CURVE ( 'NONE', #13317, #408, #21066, .T. ) ;
#127887=CIRCLE ( 'NONE', #52668, 0.1000000000000002554 ) ;
#127888=CARTESIAN_POINT ( 'NONE',  ( 12.69999999999990337, 2.500000000000000000, 3.883716857408420431 ) ) ;
#127889=DIRECTION ( 'NONE',  ( 0.000000000000000000, -0.9999939076577903929, 0.003490651415223739937 ) ) ;
#127890=DIRECTION ( 'NONE',  ( 0.000000000000000000, 1.000000000000000000, 0.000000000000000000 ) ) ;
#127891=DIRECTION ( 'NONE',  ( 0.000000000000000000, 0.000000000000000000, -1.000000000000000000 ) ) ;
#127892=CIRCLE ( 'NONE', #69389, 0.1000000000000000472 ) ;
#127893=VECTOR ( 'NONE', #100967, 1000.000000000000000 ) ;
#127894=ADVANCED_FACE ( 'NONE', ( #61660 ), #78287, .T. ) ;
#127895=EDGE_CURVE ( 'NONE', #114782, #127312, #12534, .T. ) ;
#127896=CARTESIAN_POINT ( 'NONE',  ( -5.450000000000023270, 2.500000000000000000, -2.165063509461101710 ) ) ;
#127897=EDGE_CURVE ( 'NONE', #52697, #11241, #76224, .T. ) ;
#127898=AXIS2_PLACEMENT_3D ( 'NONE', #30441, #11415, #62474 ) ;
#127899=ORIENTED_EDGE ( 'NONE', *, *, #66831, .F. ) ;
#127900=DIRECTION ( 'NONE',  ( 0.000000000000000000, 1.000000000000000000, 0.000000000000000000 ) ) ;
#127901=VERTEX_POINT ( 'NONE', #121205 ) ;
#127902=PLANE ( 'NONE',  #90193 ) ;
#127903=EDGE_CURVE ( 'NONE', #5697, #78167, #113871, .T. ) ;
#127904=VERTEX_POINT ( 'NONE', #41381 ) ;
#127905=FACE_OUTER_BOUND ( 'NONE', #38516, .T. ) ;
#127906=VECTOR ( 'NONE', #62326, 1000.000000000000000 ) ;
#127907=DIRECTION ( 'NONE',  ( 0.000000000000000000, 0.000000000000000000, 1.000000000000000000 ) ) ;
#127908=ORIENTED_EDGE ( 'NONE', *, *, #12627, .T. ) ;
#127909=DIRECTION ( 'NONE',  ( 0.000000000000000000, 0.000000000000000000, 1.000000000000000000 ) ) ;
#127910=CARTESIAN_POINT ( 'NONE',  ( 13.14999999999989733, 12.50000000000000000, -2.511473670974877948 ) ) ;
#127911=ORIENTED_EDGE ( 'NONE', *, *, #66211, .T. ) ;
#127912=EDGE_CURVE ( 'NONE', #14309, #119361, #32331, .T. ) ;
#127913=DIRECTION ( 'NONE',  ( 0.000000000000000000, 1.000000000000000000, 0.000000000000000000 ) ) ;
#127914=ORIENTED_EDGE ( 'NONE', *, *, #81120, .F. ) ;
#127915=VERTEX_POINT ( 'NONE', #42008 ) ;
#127916=DIRECTION ( 'NONE',  ( -0.000000000000000000, 1.000000000000000000, -0.000000000000000000 ) ) ;
#127919=LINE ( 'NONE', #89920, #124445 ) ;
#127920=CARTESIAN_POINT ( 'NONE',  ( -7.950000000000012612, 12.50000000000000000, 2.165063509461097713 ) ) ;
#127921=FACE_OUTER_BOUND ( 'NONE', #117783, .T. ) ;
#127922=AXIS2_PLACEMENT_3D ( 'NONE', #52793, #103186, #52157 ) ;
#127923=VECTOR ( 'NONE', #38432, 1000.000000000000000 ) ;
#127924=AXIS2_PLACEMENT_3D ( 'NONE', #19048, #86513, #47260 ) ;
#127925=VERTEX_POINT ( 'NONE', #3370 ) ;
#127926=CARTESIAN_POINT ( 'NONE',  ( -0.8500000000000382805, 2.500000000000000000, -7.188010851410854052 ) ) ;
#127927=DIRECTION ( 'NONE',  ( 0.000000000000000000, -0.9999939076577903929, 0.003490651415223739937 ) ) ;
#127928=AXIS2_PLACEMENT_3D ( 'NONE', #74196, #123291, #64365 ) ;
#127929=AXIS2_PLACEMENT_3D ( 'NONE', #85732, #85092, #64809 ) ;
#127930=AXIS2_PLACEMENT_3D ( 'NONE', #2285, #100496, #40967 ) ;
#127931=VERTEX_POINT ( 'NONE', #2716 ) ;
#127932=VECTOR ( 'NONE', #6281, 1000.000000000000000 ) ;
#127933=CONICAL_SURFACE ( 'NONE', #115379, 0.1000000000000000472, 0.003490658503988666988 ) ;
#127934=DIRECTION ( 'NONE',  ( 0.000000000000000000, 0.000000000000000000, 1.000000000000000000 ) ) ;
#127935=CARTESIAN_POINT ( 'NONE',  ( 1.649999999999949729, 2.500000000000000000, 7.088010851410848190 ) ) ;
#127936=DIRECTION ( 'NONE',  ( -0.000000000000000000, -1.000000000000000000, -0.000000000000000000 ) ) ;
#127937=CARTESIAN_POINT ( 'NONE',  ( -2.950000000000033484, 2.500000000000000000, -6.595190528383302109 ) ) ;
#127938=DIRECTION ( 'NONE',  ( 0.000000000000000000, -0.9999939076577903929, 0.003490651415223739937 ) ) ;
#127939=EDGE_LOOP ( 'NONE', ( #104243, #124043, #42541, #636 ) ) ;
#127940=AXIS2_PLACEMENT_3D ( 'NONE', #8848, #98512, #129313 ) ;
#127941=EDGE_CURVE ( 'NONE', #90263, #56748, #61560, .T. ) ;
#127942=CARTESIAN_POINT ( 'NONE',  ( 0.7999999999999548583, 12.50000000000000000, 4.265033745738159077 ) ) ;
#127943=CARTESIAN_POINT ( 'NONE',  ( -3.350000000000028955, 2.500000000000000000, 2.065063509461097624 ) ) ;
#127944=VERTEX_POINT ( 'NONE', #11894 ) ;
#127945=CARTESIAN_POINT ( 'NONE',  ( -6.050000000000020250, 2.500000000000000000, -2.511473670974877948 ) ) ;
#127946=EDGE_CURVE ( 'NONE', #113860, #47295, #101252, .T. ) ;
#127947=VERTEX_POINT ( 'NONE', #91750 ) ;
#127949=CARTESIAN_POINT ( 'NONE',  ( 8.299999999999922551, 2.500000000000000000, -4.330127018922201643 ) ) ;
#127950=VERTEX_POINT ( 'NONE', #81920 ) ;
#127952=DIRECTION ( 'NONE',  ( -4.274815082592931898E-19, -0.9999939076577903929, -0.003490651415223739937 ) ) ;
#127953=FACE_OUTER_BOUND ( 'NONE', #8053, .T. ) ;
#127954=AXIS2_PLACEMENT_3D ( 'NONE', #19407, #59378, #99282 ) ;
#127955=VERTEX_POINT ( 'NONE', #110102 ) ;
#127956=LINE ( 'NONE', #8173, #111530 ) ;
#127957=DIRECTION ( 'NONE',  ( 0.000000000000000000, 1.000000000000000000, 0.000000000000000000 ) ) ;
#127958=VERTEX_POINT ( 'NONE', #112689 ) ;
#127959=CARTESIAN_POINT ( 'NONE',  ( 1.649999999999951505, 12.50000000000000000, -2.792790559304616504 ) ) ;
#127960=DIRECTION ( 'NONE',  ( 0.000000000000000000, 0.000000000000000000, -1.000000000000000000 ) ) ;
#127961=ORIENTED_EDGE ( 'NONE', *, *, #49500, .F. ) ;
#127962=CONICAL_SURFACE ( 'NONE', #71421, 0.1000000000000000472, 0.003490658503988666988 ) ;
#127963=VECTOR ( 'NONE', #127755, 1000.000000000000000 ) ;
#127964=VECTOR ( 'NONE', #42960, 1000.000000000000000 ) ;
#127965=EDGE_LOOP ( 'NONE', ( #39448, #54473 ) ) ;
#127966=ORIENTED_EDGE ( 'NONE', *, *, #88403, .F. ) ;
#127967=DIRECTION ( 'NONE',  ( 0.000000000000000000, 0.000000000000000000, -1.000000000000000000 ) ) ;
#127968=CARTESIAN_POINT ( 'NONE',  ( -11.64999999999999680, 2.500000000000000000, -7.288010851410851032 ) ) ;
#127969=PLANE ( 'NONE',  #42232 ) ;
#127970=FACE_BOUND ( 'NONE', #129335, .T. ) ;
#127971=VERTEX_POINT ( 'NONE', #23016 ) ;
#127972=CARTESIAN_POINT ( 'NONE',  ( -5.800000000000018474, 2.500000000000000000, -2.276824562219559311E-15 ) ) ;
#127973=FACE_OUTER_BOUND ( 'NONE', #76048, .T. ) ;
#127974=AXIS2_PLACEMENT_3D ( 'NONE', #31070, #53108, #61151 ) ;
#127975=ORIENTED_EDGE ( 'NONE', *, *, #116766, .F. ) ;
#127976=AXIS2_PLACEMENT_3D ( 'NONE', #109465, #59747, #49924 ) ;
#127977=CARTESIAN_POINT ( 'NONE',  ( 5.449999999999936229, 2.500000000000000000, -2.165063509461101710 ) ) ;
#127978=EDGE_CURVE ( 'NONE', #41506, #35443, #53124, .T. ) ;
#127979=CARTESIAN_POINT ( 'NONE',  ( -8.350000000000012079, 2.500000000000000000, -1.372243186433550033 ) ) ;
#127980=AXIS2_PLACEMENT_3D ( 'NONE', #6096, #127195, #125247 ) ;
#127981=AXIS2_PLACEMENT_3D ( 'NONE', #68810, #108725, #19042 ) ;
#127983=DIRECTION ( 'NONE',  ( 0.000000000000000000, -0.9999939076577903929, 0.003490651415223739937 ) ) ;
#127984=DIRECTION ( 'NONE',  ( 0.000000000000000000, 1.000000000000000000, 0.000000000000000000 ) ) ;
#127985=CARTESIAN_POINT ( 'NONE',  ( 2.099999999999948574, 12.50000000000000000, 4.395220292106234439 ) ) ;
#127986=CARTESIAN_POINT ( 'NONE',  ( -12.69999999999999396, 2.500000000000000000, -4.083716857408424161 ) ) ;
#127987=CARTESIAN_POINT ( 'NONE',  ( -4.400000000000025224, 2.500000000000000000, 4.776537180435972196 ) ) ;
#127988=EDGE_CURVE ( 'NONE', #97598, #118985, #72023, .T. ) ;
#127989=ORIENTED_EDGE ( 'NONE', *, *, #69173, .T. ) ;
#127990=EDGE_LOOP ( 'NONE', ( #34995, #26824 ) ) ;
#127991=ORIENTED_EDGE ( 'NONE', *, *, #43113, .F. ) ;
#127992=VERTEX_POINT ( 'NONE', #100288 ) ;
#127993=EDGE_LOOP ( 'NONE', ( #103131, #129026 ) ) ;
#127994=CARTESIAN_POINT ( 'NONE',  ( -12.69999999999999041, 12.50000000000000000, 3.918623584224383727 ) ) ;
#127996=DIRECTION ( 'NONE',  ( -4.274815082592931898E-19, -0.9999939076577903929, -0.003490651415223739937 ) ) ;
#127997=ORIENTED_EDGE ( 'NONE', *, *, #48023, .F. ) ;
#127998=FACE_BOUND ( 'NONE', #40435, .T. ) ;
#127999=EDGE_CURVE ( 'NONE', #95824, #72203, #56027, .T. ) ;
#128000=CARTESIAN_POINT ( 'NONE',  ( 6.849999999999929479, 2.500000000000000000, 6.148780366869520009 ) ) ;
#128001=EDGE_CURVE ( 'NONE', #70303, #125468, #105461, .T. ) ;
#128002=FACE_OUTER_BOUND ( 'NONE', #60070, .T. ) ;
#128003=DIRECTION ( 'NONE',  ( 0.000000000000000000, 1.000000000000000000, 0.000000000000000000 ) ) ;
#128004=DIRECTION ( 'NONE',  ( 0.000000000000000000, 0.000000000000000000, 1.000000000000000000 ) ) ;
#128005=EDGE_CURVE ( 'NONE', #121848, #16531, #57434, .T. ) ;
#128006=DIRECTION ( 'NONE',  ( 0.000000000000000000, 1.000000000000000000, 0.000000000000000000 ) ) ;
#128007=EDGE_LOOP ( 'NONE', ( #28148, #73185, #102362, #120785 ) ) ;
#128008=CARTESIAN_POINT ( 'NONE',  ( 7.499999999999925393, 2.500000000000000000, -0.6928203230275541413 ) ) ;
#128009=ORIENTED_EDGE ( 'NONE', *, *, #26286, .F. ) ;
#128010=EDGE_LOOP ( 'NONE', ( #31250, #41080 ) ) ;
#128011=AXIS2_PLACEMENT_3D ( 'NONE', #110425, #91432, #40422 ) ;
#128012=EDGE_LOOP ( 'NONE', ( #109612, #95312 ) ) ;
#128013=CONICAL_SURFACE ( 'NONE', #73623, 0.1000000000000002554, 0.003490658503988666988 ) ;
#128014=DIRECTION ( 'NONE',  ( 0.000000000000000000, 0.000000000000000000, 1.000000000000000000 ) ) ;
#128015=CIRCLE ( 'NONE', #84179, 0.09999999999999982514 ) ;
#128016=CARTESIAN_POINT ( 'NONE',  ( 14.69113575804733429, 2.499999999999999112, 6.337000356224947950 ) ) ;
#128017=CARTESIAN_POINT ( 'NONE',  ( 11.89999999999990798, 2.500000000000000000, -3.983716857408426293 ) ) ;
#128018=VERTEX_POINT ( 'NONE', #84198 ) ;
#128019=DIRECTION ( 'NONE',  ( -0.000000000000000000, -1.000000000000000000, -0.000000000000000000 ) ) ;
#128020=CARTESIAN_POINT ( 'NONE',  ( 2.499999999999981792, 12.50000000000000000, 4.395220292106234439 ) ) ;
#128021=AXIS2_PLACEMENT_3D ( 'NONE', #55618, #106013, #66073 ) ;
#128022=AXIS2_PLACEMENT_3D ( 'NONE', #51633, #41823, #12960 ) ;
#128023=CIRCLE ( 'NONE', #44397, 0.1000000000000000472 ) ;
#128024=DIRECTION ( 'NONE',  ( 0.000000000000000000, 0.000000000000000000, 1.000000000000000000 ) ) ;
#128026=CARTESIAN_POINT ( 'NONE',  ( -6.249999999999984901, 2.500000000000000000, -6.395190528383301931 ) ) ;
#128027=FACE_OUTER_BOUND ( 'NONE', #24887, .T. ) ;
#128028=VECTOR ( 'NONE', #40800, 1000.000000000000000 ) ;
#128029=CONICAL_SURFACE ( 'NONE', #71589, 0.1000000000000002554, 0.003490658503988666988 ) ;
#128030=CARTESIAN_POINT ( 'NONE',  ( -5.650000000000023448, 12.50000000000000000, -6.148780366869526226 ) ) ;
#128031=VERTEX_POINT ( 'NONE', #96586 ) ;
#128032=LINE ( 'NONE', #129349, #113257 ) ;
#128033=CIRCLE ( 'NONE', #67355, 0.06509327318403745899 ) ;
#128034=VERTEX_POINT ( 'NONE', #124129 ) ;
#128035=EDGE_CURVE ( 'NONE', #26403, #69417, #6908, .T. ) ;
#128036=ORIENTED_EDGE ( 'NONE', *, *, #16426, .T. ) ;
#128037=CARTESIAN_POINT ( 'NONE',  ( -11.44999999999999751, 2.500000000000000000, 6.841600689897072485 ) ) ;
#128038=LINE ( 'NONE', #27903, #107327 ) ;
#128039=CARTESIAN_POINT ( 'NONE',  ( 13.74999999999989697, 2.500000000000000000, 2.857883832488649301 ) ) ;
#128040=EDGE_LOOP ( 'NONE', ( #7137, #36840 ) ) ;
#128042=ADVANCED_FACE ( 'NONE', ( #34485 ), #115913, .T. ) ;
#128043=AXIS2_PLACEMENT_3D ( 'NONE', #97355, #48255, #67213 ) ;
#128044=DIRECTION ( 'NONE',  ( 0.000000000000000000, -0.9999939076577903929, 0.003490651415223739937 ) ) ;
#128045=CARTESIAN_POINT ( 'NONE',  ( 3.749999999999938716, 12.50000000000000000, 7.188010851410848723 ) ) ;
#128046=DIRECTION ( 'NONE',  ( 0.000000000000000000, 1.000000000000000000, 0.000000000000000000 ) ) ;
#128047=ORIENTED_EDGE ( 'NONE', *, *, #20125, .F. ) ;
#128048=ORIENTED_EDGE ( 'NONE', *, *, #100581, .F. ) ;
#128049=EDGE_CURVE ( 'NONE', #31868, #31765, #105129, .T. ) ;
#128050=CARTESIAN_POINT ( 'NONE',  ( -13.09999999999999254, 2.500000000000000000, -3.983716857408423628 ) ) ;
#128052=EDGE_CURVE ( 'NONE', #70878, #99834, #28099, .T. ) ;
#128053=CONICAL_SURFACE ( 'NONE', #84122, 0.09999999999999982514, 0.003490658503988666988 ) ;
#128054=EDGE_LOOP ( 'NONE', ( #81280, #56323 ) ) ;
#128055=DIRECTION ( 'NONE',  ( 0.000000000000000000, 0.000000000000000000, 1.000000000000000000 ) ) ;
#128056=AXIS2_PLACEMENT_3D ( 'NONE', #21096, #13199, #32879 ) ;
#128057=DIRECTION ( 'NONE',  ( 0.000000000000000000, 1.000000000000000000, 0.000000000000000000 ) ) ;
#128058=EDGE_LOOP ( 'NONE', ( #109172, #41879, #7317, #104479 ) ) ;
#128059=CARTESIAN_POINT ( 'NONE',  ( -8.950000000000004619, 12.50000000000000000, 6.213873640053559022 ) ) ;
#128060=EDGE_CURVE ( 'NONE', #2830, #57084, #69963, .T. ) ;
#128061=DIRECTION ( 'NONE',  ( 0.000000000000000000, -0.000000000000000000, 1.000000000000000000 ) ) ;
#128063=DIRECTION ( 'NONE',  ( 0.000000000000000000, 0.000000000000000000, 1.000000000000000000 ) ) ;
#128064=CIRCLE ( 'NONE', #40231, 0.06509327318403743123 ) ;
#128065=EDGE_LOOP ( 'NONE', ( #94223, #36540, #40953, #70013 ) ) ;
#128066=VECTOR ( 'NONE', #36939, 1000.000000000000000 ) ;
#128067=EDGE_CURVE ( 'NONE', #13197, #59055, #80431, .T. ) ;
#128068=CIRCLE ( 'NONE', #107115, 0.1000000000000002554 ) ;
#128069=CARTESIAN_POINT ( 'NONE',  ( -3.350000000000028511, 2.500000000000000000, -2.857883832488653741 ) ) ;
#128070=ADVANCED_FACE ( 'NONE', ( #44938 ), #15554, .T. ) ;
#128071=CONICAL_SURFACE ( 'NONE', #19380, 0.1000000000000002554, 0.003490658503988666988 ) ;
#128072=ORIENTED_EDGE ( 'NONE', *, *, #116653, .F. ) ;
#128073=VERTEX_POINT ( 'NONE', #86777 ) ;
#128074=DIRECTION ( 'NONE',  ( 0.000000000000000000, -0.9999939076577903929, 0.003490651415223739937 ) ) ;
#128075=PLANE ( 'NONE',  #84659 ) ;
#128076=LINE ( 'NONE', #17451, #90749 ) ;
#128077=DIRECTION ( 'NONE',  ( 0.000000000000000000, 0.000000000000000000, 1.000000000000000000 ) ) ;
#128078=DIRECTION ( 'NONE',  ( 0.000000000000000000, -0.9999939076577903929, 0.003490651415223739937 ) ) ;
#128079=DIRECTION ( 'NONE',  ( 0.000000000000000000, 1.000000000000000000, 0.000000000000000000 ) ) ;
#128080=AXIS2_PLACEMENT_3D ( 'NONE', #19651, #119135, #89675 ) ;
#128081=CARTESIAN_POINT ( 'NONE',  ( 6.849999999999929479, 2.500000000000000000, -1.918653347947326004 ) ) ;
#128083=FACE_OUTER_BOUND ( 'NONE', #38739, .T. ) ;
#128084=AXIS2_PLACEMENT_3D ( 'NONE', #82183, #13426, #101825 ) ;
#128085=AXIS2_PLACEMENT_3D ( 'NONE', #24196, #66041, #14351 ) ;
#128086=DIRECTION ( 'NONE',  ( 0.000000000000000000, 0.000000000000000000, 1.000000000000000000 ) ) ;
#128087=CONICAL_SURFACE ( 'NONE', #88345, 0.1000000000000002554, 0.003490658503988666988 ) ;
#128088=FACE_OUTER_BOUND ( 'NONE', #70209, .T. ) ;
#128089=CIRCLE ( 'NONE', #31955, 0.1000000000000002554 ) ;
#128090=ORIENTED_EDGE ( 'NONE', *, *, #120257, .T. ) ;
#128091=DIRECTION ( 'NONE',  ( 0.000000000000000000, 0.000000000000000000, 1.000000000000000000 ) ) ;
#128092=DIRECTION ( 'NONE',  ( 0.000000000000000000, 1.000000000000000000, 0.000000000000000000 ) ) ;
#128093=DIRECTION ( 'NONE',  ( 0.000000000000000000, 0.000000000000000000, 1.000000000000000000 ) ) ;
#128094=DIRECTION ( 'NONE',  ( 0.000000000000000000, 0.000000000000000000, 1.000000000000000000 ) ) ;
#128095=DIRECTION ( 'NONE',  ( -0.000000000000000000, 1.000000000000000000, -0.000000000000000000 ) ) ;
#128096=VERTEX_POINT ( 'NONE', #16090 ) ;
#128097=DIRECTION ( 'NONE',  ( -0.000000000000000000, 1.000000000000000000, -0.000000000000000000 ) ) ;
#128099=DIRECTION ( 'NONE',  ( 0.000000000000000000, 1.000000000000000000, 0.000000000000000000 ) ) ;
#128100=ORIENTED_EDGE ( 'NONE', *, *, #83305, .T. ) ;
#128101=AXIS2_PLACEMENT_3D ( 'NONE', #110027, #9884, #119194 ) ;
#128102=CIRCLE ( 'NONE', #86313, 0.06509327318403745899 ) ;
#128103=VERTEX_POINT ( 'NONE', #37060 ) ;
#128104=DIRECTION ( 'NONE',  ( 0.000000000000000000, -0.000000000000000000, 1.000000000000000000 ) ) ;
#128105=EDGE_CURVE ( 'NONE', #16630, #109444, #109669, .T. ) ;
#128106=ORIENTED_EDGE ( 'NONE', *, *, #35914, .T. ) ;
#128107=ORIENTED_EDGE ( 'NONE', *, *, #106153, .F. ) ;
#128108=AXIS2_PLACEMENT_3D ( 'NONE', #56005, #66474, #96569 ) ;
#128109=ORIENTED_EDGE ( 'NONE', *, *, #125363, .F. ) ;
#128110=DIRECTION ( 'NONE',  ( 0.000000000000000000, 1.000000000000000000, 0.000000000000000000 ) ) ;
#128111=AXIS2_PLACEMENT_3D ( 'NONE', #34719, #74617, #114527 ) ;
#128112=CARTESIAN_POINT ( 'NONE',  ( -12.89999999999999325, 12.50000000000000000, 0.6928203230275535862 ) ) ;
#128113=CARTESIAN_POINT ( 'NONE',  ( -10.65000000000000391, 2.500000000000000000, -6.148780366869522673 ) ) ;
#128114=CARTESIAN_POINT ( 'NONE',  ( 12.09999999999990195, 2.500000000000000000, 0.7928203230275495672 ) ) ;
#128115=AXIS2_PLACEMENT_3D ( 'NONE', #30881, #70781, #91068 ) ;
#128116=ORIENTED_EDGE ( 'NONE', *, *, #108057, .F. ) ;
#128117=CONICAL_SURFACE ( 'NONE', #115567, 0.1000000000000000472, 0.003490658503988666988 ) ;
#128118=AXIS2_PLACEMENT_3D ( 'NONE', #18612, #250, #118744 ) ;
#128119=CARTESIAN_POINT ( 'NONE',  ( -8.950000000000008171, 12.50000000000000000, -2.511473670974877948 ) ) ;
#128121=ORIENTED_EDGE ( 'NONE', *, *, #122697, .F. ) ;
#128122=DIRECTION ( 'NONE',  ( 0.000000000000000000, 0.000000000000000000, 1.000000000000000000 ) ) ;
#128123=DIRECTION ( 'NONE',  ( 0.000000000000000000, 0.000000000000000000, 1.000000000000000000 ) ) ;
#128124=AXIS2_PLACEMENT_3D ( 'NONE', #3130, #71214, #21475 ) ;
#128125=CARTESIAN_POINT ( 'NONE',  ( 15.05551045036142277, 2.483581587658090228, 4.666934263335511091 ) ) ;
#128126=DIRECTION ( 'NONE',  ( 0.000000000000000000, -0.9999939076577903929, 0.003490651415223739937 ) ) ;
#128127=CARTESIAN_POINT ( 'NONE',  ( 4.149999999999941735, 12.50000000000000000, -2.792790559304616504 ) ) ;
#128128=CONICAL_SURFACE ( 'NONE', #52812, 0.09999999999999999167, 0.003490658503988666988 ) ;
#128129=ORIENTED_EDGE ( 'NONE', *, *, #56798, .F. ) ;
#128130=ORIENTED_EDGE ( 'NONE', *, *, #114965, .F. ) ;
#128131=EDGE_LOOP ( 'NONE', ( #18180, #127767 ) ) ;
#128132=ORIENTED_EDGE ( 'NONE', *, *, #75766, .T. ) ;
#128133=ORIENTED_EDGE ( 'NONE', *, *, #69952, .T. ) ;
#128134=DIRECTION ( 'NONE',  ( 0.000000000000000000, 1.000000000000000000, 0.000000000000000000 ) ) ;
#128135=CARTESIAN_POINT ( 'NONE',  ( 43.31340625566036096, 2.029328411521368558, 5.113049425667499648 ) ) ;
#128136=CARTESIAN_POINT ( 'NONE',  ( 10.39999999999991154, 2.500000000000000000, -3.637306695894650055 ) ) ;
#128137=FACE_BOUND ( 'NONE', #32755, .T. ) ;
#128138=FACE_OUTER_BOUND ( 'NONE', #101500, .T. ) ;
#128139=CARTESIAN_POINT ( 'NONE',  ( -5.850000000000018296, 2.500000000000000000, 1.572243186433545548 ) ) ;
#128140=FACE_OUTER_BOUND ( 'NONE', #107089, .T. ) ;
#128141=DIRECTION ( 'NONE',  ( 0.000000000000000000, -0.9999939076577903929, 0.003490651415223739937 ) ) ;
#128142=AXIS2_PLACEMENT_3D ( 'NONE', #30424, #80803, #110248 ) ;
#128143=DIRECTION ( 'NONE',  ( -4.274815082592931898E-19, -0.9999939076577903929, -0.003490651415223739937 ) ) ;
#128146=CIRCLE ( 'NONE', #21534, 0.06509327318403745899 ) ;
#128147=CIRCLE ( 'NONE', #23783, 0.06509327318403745899 ) ;
#128148=EDGE_CURVE ( 'NONE', #38872, #116591, #67797, .T. ) ;
#128149=DIRECTION ( 'NONE',  ( 0.000000000000000000, 1.000000000000000000, 0.000000000000000000 ) ) ;
#128150=VERTEX_POINT ( 'NONE', #126719 ) ;
#128151=ORIENTED_EDGE ( 'NONE', *, *, #15615, .T. ) ;
#128152=ORIENTED_EDGE ( 'NONE', *, *, #94490, .F. ) ;
#128154=ADVANCED_FACE ( 'NONE', ( #4988 ), #34463, .T. ) ;
#128155=LINE ( 'NONE', #129472, #123955 ) ;
#128156=FACE_BOUND ( 'NONE', #59823, .T. ) ;
#128157=CIRCLE ( 'NONE', #40339, 0.06509327318403745899 ) ;
#128158=EDGE_CURVE ( 'NONE', #68530, #73774, #25267, .T. ) ;
#128159=AXIS2_PLACEMENT_3D ( 'NONE', #119676, #109875, #38576 ) ;
#128160=DIRECTION ( 'NONE',  ( 0.000000000000000000, 1.000000000000000000, 0.000000000000000000 ) ) ;
#128161=AXIS2_PLACEMENT_3D ( 'NONE', #109339, #90990, #9858 ) ;
#128162=VECTOR ( 'NONE', #8619, 1000.000000000000000 ) ;
#128163=EDGE_CURVE ( 'NONE', #73692, #14356, #34376, .T. ) ;
#128164=ADVANCED_FACE ( 'NONE', ( #17380 ), #59522, .T. ) ;
#128166=FACE_OUTER_BOUND ( 'NONE', #91629, .T. ) ;
#128167=LINE ( 'NONE', #28678, #1333 ) ;
#128168=FACE_OUTER_BOUND ( 'NONE', #48367, .T. ) ;
#128169=EDGE_CURVE ( 'NONE', #83800, #8589, #74166, .T. ) ;
#128170=DIRECTION ( 'NONE',  ( 0.000000000000000000, 1.000000000000000000, 0.000000000000000000 ) ) ;
#128171=ORIENTED_EDGE ( 'NONE', *, *, #26649, .F. ) ;
#128172=DIRECTION ( 'NONE',  ( 0.000000000000000000, -0.9999939076577903929, 0.003490651415223739937 ) ) ;
#128173=LINE ( 'NONE', #109149, #120213 ) ;
#128174=AXIS2_PLACEMENT_3D ( 'NONE', #47736, #66066, #106004 ) ;
#128175=CONICAL_SURFACE ( 'NONE', #71741, 0.1000000000000002554, 0.003490658503988666988 ) ;
#128176=VERTEX_POINT ( 'NONE', #10168 ) ;
#128178=FACE_OUTER_BOUND ( 'NONE', #72223, .T. ) ;
#128179=DIRECTION ( 'NONE',  ( -4.274815082592931898E-19, -0.9999939076577903929, -0.003490651415223739937 ) ) ;
#128180=AXIS2_PLACEMENT_3D ( 'NONE', #81619, #51537, #82282 ) ;
#128181=ORIENTED_EDGE ( 'NONE', *, *, #30254, .F. ) ;
#128182=DIRECTION ( 'NONE',  ( -4.274815082592931898E-19, -0.9999939076577903929, -0.003490651415223739937 ) ) ;
#128183=VECTOR ( 'NONE', #34179, 1000.000000000000000 ) ;
#128184=LINE ( 'NONE', #45756, #83255 ) ;
#128185=ORIENTED_EDGE ( 'NONE', *, *, #56487, .T. ) ;
#128186=CARTESIAN_POINT ( 'NONE',  ( -9.350000000000004974, 12.50000000000000000, 6.213873640053559022 ) ) ;
#128187=ORIENTED_EDGE ( 'NONE', *, *, #10966, .T. ) ;
#128188=DIRECTION ( 'NONE',  ( -0.000000000000000000, 1.000000000000000000, -0.000000000000000000 ) ) ;
#128189=ORIENTED_EDGE ( 'NONE', *, *, #115763, .F. ) ;
#128190=DIRECTION ( 'NONE',  ( 0.000000000000000000, -0.000000000000000000, 1.000000000000000000 ) ) ;
#128191=FACE_BOUND ( 'NONE', #60284, .T. ) ;
#128192=VERTEX_POINT ( 'NONE', #87422 ) ;
#128194=ORIENTED_EDGE ( 'NONE', *, *, #66576, .T. ) ;
#128195=DIRECTION ( 'NONE',  ( 0.000000000000000000, 0.000000000000000000, -1.000000000000000000 ) ) ;
#128196=DIRECTION ( 'NONE',  ( -4.274815082592931898E-19, -0.9999939076577903929, -0.003490651415223739937 ) ) ;
#128197=DIRECTION ( 'NONE',  ( 0.000000000000000000, 1.000000000000000000, 0.000000000000000000 ) ) ;
#128198=CIRCLE ( 'NONE', #96875, 0.1000000000000002554 ) ;
#128199=EDGE_CURVE ( 'NONE', #109355, #25435, #86671, .T. ) ;
#128201=CARTESIAN_POINT ( 'NONE',  ( 17.50000000000000711, 2.499999999999961808, -3.093175630837484924 ) ) ;
#128202=ORIENTED_EDGE ( 'NONE', *, *, #68787, .F. ) ;
#128203=EDGE_LOOP ( 'NONE', ( #31454, #84225 ) ) ;
#128204=ORIENTED_EDGE ( 'NONE', *, *, #994, .T. ) ;
#128205=CARTESIAN_POINT ( 'NONE',  ( 10.59999999999990905, 2.500000000000000000, 3.983716857408420076 ) ) ;
#128206=VECTOR ( 'NONE', #22680, 1000.000000000000000 ) ;
#128207=VECTOR ( 'NONE', #118480, 1000.000000000000000 ) ;
#128208=CARTESIAN_POINT ( 'NONE',  ( -11.89999999999999503, 2.500000000000000000, 4.083716857408420609 ) ) ;
#128209=CIRCLE ( 'NONE', #61308, 0.1000000000000002554 ) ;
#128210=AXIS2_PLACEMENT_3D ( 'NONE', #66406, #27139, #57901 ) ;
#128211=CARTESIAN_POINT ( 'NONE',  ( 5.199999999999933564, 12.50000000000000000, 4.048810130592458201 ) ) ;
#128212=ADVANCED_FACE ( 'NONE', ( #80203 ), #46978, .T. ) ;
#128213=ORIENTED_EDGE ( 'NONE', *, *, #66472, .F. ) ;
#128214=ORIENTED_EDGE ( 'NONE', *, *, #21014, .F. ) ;
#128215=VERTEX_POINT ( 'NONE', #39013 ) ;
#128216=EDGE_CURVE ( 'NONE', #45538, #94583, #103408, .T. ) ;
#128217=DIRECTION ( 'NONE',  ( 0.000000000000000000, 0.000000000000000000, 1.000000000000000000 ) ) ;
#128219=FACE_OUTER_BOUND ( 'NONE', #108857, .T. ) ;
#128220=CIRCLE ( 'NONE', #86425, 0.09999999999999982514 ) ;
#128221=AXIS2_PLACEMENT_3D ( 'NONE', #90514, #100353, #100985 ) ;
#128222=AXIS2_PLACEMENT_3D ( 'NONE', #112803, #42126, #1541 ) ;
#128223=CARTESIAN_POINT ( 'NONE',  ( -12.49999999999995914, 12.50000000000000000, -0.06509327318403558549 ) ) ;
#128224=DIRECTION ( 'NONE',  ( -0.000000000000000000, -1.000000000000000000, -0.000000000000000000 ) ) ;
#128225=CARTESIAN_POINT ( 'NONE',  ( -1.050000000000038236, 2.500000000000000000, -1.818653347947326138 ) ) ;
#128226=CARTESIAN_POINT ( 'NONE',  ( 6.649999999999930189, 2.500000000000000000, -2.857883832488653741 ) ) ;
#128227=DIRECTION ( 'NONE',  ( -0.000000000000000000, -1.000000000000000000, -0.000000000000000000 ) ) ;
#128228=EDGE_CURVE ( 'NONE', #11179, #16737, #118064, .T. ) ;
#128229=CONICAL_SURFACE ( 'NONE', #92707, 0.09999999999999982514, 0.003490658503988666988 ) ;
#128230=EDGE_CURVE ( 'NONE', #71603, #46014, #78924, .T. ) ;
#128231=DIRECTION ( 'NONE',  ( -4.274815082592931898E-19, -0.9999939076577903929, -0.003490651415223739937 ) ) ;
#128232=AXIS2_PLACEMENT_3D ( 'NONE', #71392, #30222, #99596 ) ;
#128233=ADVANCED_FACE ( 'NONE', ( #37697 ), #9414, .T. ) ;
#128234=ORIENTED_EDGE ( 'NONE', *, *, #18824, .F. ) ;
#128235=ADVANCED_FACE ( 'NONE', ( #50109 ), #109758, .T. ) ;
#128236=ORIENTED_EDGE ( 'NONE', *, *, #599, .F. ) ;
#128237=FACE_OUTER_BOUND ( 'NONE', #19215, .T. ) ;
#128238=ADVANCED_FACE ( 'NONE', ( #128002 ), #57984, .T. ) ;
#128239=DIRECTION ( 'NONE',  ( 0.000000000000000000, 1.000000000000000000, 0.000000000000000000 ) ) ;
#128240=ORIENTED_EDGE ( 'NONE', *, *, #60971, .T. ) ;
#128241=VERTEX_POINT ( 'NONE', #8219 ) ;
#128243=DIRECTION ( 'NONE',  ( 0.000000000000000000, -0.9999939076577903929, 0.003490651415223739937 ) ) ;
#128244=DIRECTION ( 'NONE',  ( 0.000000000000000000, -0.000000000000000000, 1.000000000000000000 ) ) ;
#128245=EDGE_CURVE ( 'NONE', #74234, #116433, #82579, .T. ) ;
#128246=AXIS2_PLACEMENT_3D ( 'NONE', #17163, #97688, #45388 ) ;
#128247=CARTESIAN_POINT ( 'NONE',  ( -0.8500000000000395017, 2.500000000000000000, 6.395190528383296602 ) ) ;
#128248=CARTESIAN_POINT ( 'NONE',  ( 1.649999999999948841, 2.500000000000000000, 6.495190528383297135 ) ) ;
#128249=CARTESIAN_POINT ( 'NONE',  ( 8.099999999999921485, 12.50000000000000000, 0.3464101615137735735 ) ) ;
#128250=FACE_OUTER_BOUND ( 'NONE', #77338, .T. ) ;
#128251=CIRCLE ( 'NONE', #46668, 0.06509327318403745899 ) ;
#128252=FACE_OUTER_BOUND ( 'NONE', #31918, .T. ) ;
#128253=CIRCLE ( 'NONE', #19468, 0.06509327318403741736 ) ;
#128255=ORIENTED_EDGE ( 'NONE', *, *, #127310, .F. ) ;
#128256=EDGE_LOOP ( 'NONE', ( #128940, #102384 ) ) ;
#128257=VERTEX_POINT ( 'NONE', #88722 ) ;
#128258=ADVANCED_FACE ( 'NONE', ( #109657 ), #78375, .T. ) ;
#128259=ORIENTED_EDGE ( 'NONE', *, *, #116089, .T. ) ;
#128260=CONICAL_SURFACE ( 'NONE', #29963, 0.1000000000000000472, 0.003490658503988666988 ) ;
#128261=CARTESIAN_POINT ( 'NONE',  ( 11.64999999999990621, 12.50000000000000000, 6.495190528383297135 ) ) ;
#128262=CARTESIAN_POINT ( 'NONE',  ( -5.000000000000022204, 2.500000000000000000, 3.637306695894644726 ) ) ;
#128263=CONICAL_SURFACE ( 'NONE', #119835, 0.09999999999999982514, 0.003490658503988666988 ) ;
#128265=VERTEX_POINT ( 'NONE', #59933 ) ;
#128266=DIRECTION ( 'NONE',  ( -4.274815082592931898E-19, -0.9999939076577903929, -0.003490651415223739937 ) ) ;
#128267=CIRCLE ( 'NONE', #32127, 0.09999999999999982514 ) ;
#128268=CARTESIAN_POINT ( 'NONE',  ( 17.50000000000000000, -2.750000000000000444, -3.999999999999998224 ) ) ;
#128269=CARTESIAN_POINT ( 'NONE',  ( 8.749999999999953815, 2.500000000000000000, -2.165063509461101710 ) ) ;
#128270=CARTESIAN_POINT ( 'NONE',  ( 9.349999999999919709, 12.50000000000000000, 1.818653347947321475 ) ) ;
#128271=ORIENTED_EDGE ( 'NONE', *, *, #9847, .F. ) ;
#128273=PLANE ( 'NONE',  #20710 ) ;
#128274=ORIENTED_EDGE ( 'NONE', *, *, #99872, .F. ) ;
#128275=ADVANCED_FACE ( 'NONE', ( #77598 ), #55379, .T. ) ;
#128276=VECTOR ( 'NONE', #29757, 1000.000000000000000 ) ;
#128277=CIRCLE ( 'NONE', #98922, 0.1000000000000002554 ) ;
#128278=CONICAL_SURFACE ( 'NONE', #25861, 0.1000000000000000472, 0.003490658503988666988 ) ;
#128279=EDGE_LOOP ( 'NONE', ( #89264, #111859, #57320, #119780 ) ) ;
#128280=ORIENTED_EDGE ( 'NONE', *, *, #120186, .T. ) ;
#128281=DIRECTION ( 'NONE',  ( 0.000000000000000000, 0.000000000000000000, 1.000000000000000000 ) ) ;
#128282=DIRECTION ( 'NONE',  ( 0.000000000000000000, 0.000000000000000000, 1.000000000000000000 ) ) ;
#128283=VECTOR ( 'NONE', #67596, 1000.000000000000000 ) ;
#128284=VERTEX_POINT ( 'NONE', #8853 ) ;
#128285=CARTESIAN_POINT ( 'NONE',  ( -13.09999999999999254, 12.50000000000000000, -3.983716857408423628 ) ) ;
#128286=FACE_OUTER_BOUND ( 'NONE', #98196, .T. ) ;
#128287=EDGE_CURVE ( 'NONE', #77998, #45135, #103498, .T. ) ;
#128288=CARTESIAN_POINT ( 'NONE',  ( 7.699999999999922018, 12.50000000000000000, 0.2813168883297361700 ) ) ;
#128289=FACE_OUTER_BOUND ( 'NONE', #6939, .T. ) ;
#128290=ORIENTED_EDGE ( 'NONE', *, *, #121066, .T. ) ;
#128291=CARTESIAN_POINT ( 'NONE',  ( -1.650000000000035216, 12.50000000000000000, -1.472243186433550122 ) ) ;
#128292=ORIENTED_EDGE ( 'NONE', *, *, #100439, .T. ) ;
#128293=ORIENTED_EDGE ( 'NONE', *, *, #10990, .T. ) ;
#128294=CARTESIAN_POINT ( 'NONE',  ( -7.900000000000014566, 12.50000000000000000, -0.06509327318403970719 ) ) ;
#128295=AXIS2_PLACEMENT_3D ( 'NONE', #101982, #123533, #32626 ) ;
#128296=CIRCLE ( 'NONE', #71858, 0.06509327318403745899 ) ;
#128297=DIRECTION ( 'NONE',  ( 0.000000000000000000, -0.9999939076577903929, 0.003490651415223739937 ) ) ;
#128298=FACE_BOUND ( 'NONE', #33566, .T. ) ;
#128299=LINE ( 'NONE', #38642, #63866 ) ;
#128300=CARTESIAN_POINT ( 'NONE',  ( -7.900000000000014566, 12.50000000000000000, -4.330127018922201643 ) ) ;
#128301=DIRECTION ( 'NONE',  ( 0.000000000000000000, -0.000000000000000000, 1.000000000000000000 ) ) ;
#128302=AXIS2_PLACEMENT_3D ( 'NONE', #41532, #80148, #60523 ) ;
#128303=VECTOR ( 'NONE', #65272, 1000.000000000000000 ) ;
#128304=VECTOR ( 'NONE', #77749, 1000.000000000000000 ) ;
#128305=AXIS2_PLACEMENT_3D ( 'NONE', #77001, #46905, #116908 ) ;
#128306=CIRCLE ( 'NONE', #57189, 0.1000000000000002554 ) ;
#128307=EDGE_LOOP ( 'NONE', ( #120771, #84355 ) ) ;
#128309=DIRECTION ( 'NONE',  ( 0.000000000000000000, 1.000000000000000000, 0.000000000000000000 ) ) ;
#128310=DIRECTION ( 'NONE',  ( -4.274815082592931898E-19, -0.9999939076577903929, -0.003490651415223739937 ) ) ;
#128312=ORIENTED_EDGE ( 'NONE', *, *, #95051, .T. ) ;
#128313=AXIS2_PLACEMENT_3D ( 'NONE', #79181, #108617, #49079 ) ;
#128314=CARTESIAN_POINT ( 'NONE',  ( 8.549999999999922551, 12.50000000000000000, -6.148780366869526226 ) ) ;
#128315=AXIS2_PLACEMENT_3D ( 'NONE', #32278, #93116, #22454 ) ;
#128316=AXIS2_PLACEMENT_3D ( 'NONE', #124609, #34954, #56494 ) ;
#128317=EDGE_CURVE ( 'NONE', #4728, #113637, #51292, .T. ) ;
#128318=LINE ( 'NONE', #58917, #11854 ) ;
#128319=VERTEX_POINT ( 'NONE', #29175 ) ;
#128320=ORIENTED_EDGE ( 'NONE', *, *, #121474, .F. ) ;
#128321=CONICAL_SURFACE ( 'NONE', #88598, 0.1000000000000002554, 0.003490658503988666988 ) ;
#128322=CARTESIAN_POINT ( 'NONE',  ( -3.350000000000028955, 2.500000000000000000, 5.802370205355744659 ) ) ;
#128323=DIRECTION ( 'NONE',  ( -0.000000000000000000, -1.000000000000000000, -0.000000000000000000 ) ) ;
#128324=FACE_BOUND ( 'NONE', #39900, .T. ) ;
#128325=EDGE_CURVE ( 'NONE', #123030, #35541, #23194, .T. ) ;
#128326=CARTESIAN_POINT ( 'NONE',  ( 12.30568799055497564, -2.500000000000000444, -7.490555763477718898 ) ) ;
#128327=EDGE_LOOP ( 'NONE', ( #20154, #66270, #105597, #92394 ) ) ;
#128328=DIRECTION ( 'NONE',  ( 0.000000000000000000, 0.000000000000000000, -1.000000000000000000 ) ) ;
#128329=EDGE_CURVE ( 'NONE', #25124, #97893, #62506, .T. ) ;
#128330=ORIENTED_EDGE ( 'NONE', *, *, #11734, .F. ) ;
#128331=EDGE_CURVE ( 'NONE', #102405, #47378, #67883, .T. ) ;
#128332=ORIENTED_EDGE ( 'NONE', *, *, #80926, .T. ) ;
#128333=CARTESIAN_POINT ( 'NONE',  ( -10.60000000000000142, 2.500000000000000000, 4.576537180435972019 ) ) ;
#128334=EDGE_CURVE ( 'NONE', #82736, #21628, #70048, .T. ) ;
#128335=ADVANCED_FACE ( 'NONE', ( #71024 ), #111823, .T. ) ;
#128337=ADVANCED_FACE ( 'NONE', ( #120763 ), #10773, .T. ) ;
#128339=EDGE_LOOP ( 'NONE', ( #48999, #14910 ) ) ;
#128340=CARTESIAN_POINT ( 'NONE',  ( -9.600000000000008527, 12.50000000000000000, -3.572213422710607933 ) ) ;
#128341=DIRECTION ( 'NONE',  ( 0.000000000000000000, 1.000000000000000000, 0.000000000000000000 ) ) ;
#128342=DIRECTION ( 'NONE',  ( 0.000000000000000000, 1.000000000000000000, 0.000000000000000000 ) ) ;
#128343=PLANE ( 'NONE',  #69769 ) ;
#128344=ADVANCED_FACE ( 'NONE', ( #102416 ), #40828, .T. ) ;
#128345=CIRCLE ( 'NONE', #775, 0.06509327318403743123 ) ;
#128346=VECTOR ( 'NONE', #94331, 1000.000000000000000 ) ;
#128347=EDGE_CURVE ( 'NONE', #53973, #60435, #105559, .T. ) ;
#128348=EDGE_CURVE ( 'NONE', #30682, #107108, #76309, .T. ) ;
#128349=ORIENTED_EDGE ( 'NONE', *, *, #66839, .T. ) ;
#128350=DIRECTION ( 'NONE',  ( 0.000000000000000000, 0.000000000000000000, 1.000000000000000000 ) ) ;
#128351=DIRECTION ( 'NONE',  ( -0.000000000000000000, -1.000000000000000000, -0.000000000000000000 ) ) ;
#128352=PLANE ( 'NONE',  #74316 ) ;
#128354=ORIENTED_EDGE ( 'NONE', *, *, #121529, .T. ) ;
#128355=DIRECTION ( 'NONE',  ( 0.000000000000000000, -0.9999939076577903929, 0.003490651415223739937 ) ) ;
#128356=ORIENTED_EDGE ( 'NONE', *, *, #7889, .F. ) ;
#128357=AXIS2_PLACEMENT_3D ( 'NONE', #2383, #62634, #102536 ) ;
#128358=DIRECTION ( 'NONE',  ( 0.000000000000000000, 1.000000000000000000, 0.000000000000000000 ) ) ;
#128359=VERTEX_POINT ( 'NONE', #110923 ) ;
#128360=AXIS2_PLACEMENT_3D ( 'NONE', #80225, #20017, #99866 ) ;
#128361=DIRECTION ( 'NONE',  ( 0.000000000000000000, 0.000000000000000000, 1.000000000000000000 ) ) ;
#128362=DIRECTION ( 'NONE',  ( -0.000000000000000000, 1.000000000000000000, -0.000000000000000000 ) ) ;
#128365=DIRECTION ( 'NONE',  ( 0.000000000000000000, -0.9999939076577903929, 0.003490651415223739937 ) ) ;
#128366=ORIENTED_EDGE ( 'NONE', *, *, #14185, .F. ) ;
#128367=DIRECTION ( 'NONE',  ( 0.000000000000000000, 1.000000000000000000, 0.000000000000000000 ) ) ;
#128368=FACE_OUTER_BOUND ( 'NONE', #93193, .T. ) ;
#128370=DIRECTION ( 'NONE',  ( 0.000000000000000000, 0.000000000000000000, 1.000000000000000000 ) ) ;
#128371=CARTESIAN_POINT ( 'NONE',  ( -8.150000000000009237, 2.500000000000000000, 6.248780366869520542 ) ) ;
#128372=CARTESIAN_POINT ( 'NONE',  ( -12.89999999999999147, 12.50000000000000000, -5.022947341949751454 ) ) ;
#128373=ORIENTED_EDGE ( 'NONE', *, *, #111197, .T. ) ;
#128374=EDGE_LOOP ( 'NONE', ( #73388, #95090 ) ) ;
#128375=CARTESIAN_POINT ( 'NONE',  ( 9.599999999999914380, 2.500000000000000000, 5.022947341949748790 ) ) ;
#128376=AXIS2_PLACEMENT_3D ( 'NONE', #126, #99640, #39456 ) ;
#128377=ORIENTED_EDGE ( 'NONE', *, *, #124484, .T. ) ;
#128378=CONICAL_SURFACE ( 'NONE', #76030, 0.09999999999999982514, 0.003490658503988666988 ) ;
#128379=CIRCLE ( 'NONE', #71932, 0.06509327318403745899 ) ;
#128380=CARTESIAN_POINT ( 'NONE',  ( 8.099999999999923261, 12.50000000000000000, -4.676537180435978769 ) ) ;
#128381=ORIENTED_EDGE ( 'NONE', *, *, #41588, .T. ) ;
#128382=ORIENTED_EDGE ( 'NONE', *, *, #47768, .F. ) ;
#128383=VERTEX_POINT ( 'NONE', #82125 ) ;
#128384=CIRCLE ( 'NONE', #82406, 0.06509327318403745899 ) ;
#128385=CARTESIAN_POINT ( 'NONE',  ( 87.50000000000001421, 3.413194297214863671, -6.711110875543777610 ) ) ;
#128386=AXIS2_PLACEMENT_3D ( 'NONE', #53452, #122828, #101899 ) ;
#128387=DIRECTION ( 'NONE',  ( -0.000000000000000000, -1.000000000000000000, -0.000000000000000000 ) ) ;
#128388=LINE ( 'NONE', #107431, #60216 ) ;
#128390=DIRECTION ( 'NONE',  ( 0.000000000000000000, 0.000000000000000000, -1.000000000000000000 ) ) ;
#128391=DIRECTION ( 'NONE',  ( 0.000000000000000000, 1.000000000000000000, 0.000000000000000000 ) ) ;
#128392=CARTESIAN_POINT ( 'NONE',  ( 8.949999999999915801, 2.500000000000000000, 6.941600689897073018 ) ) ;
#128393=ADVANCED_FACE ( 'NONE', ( #2931 ), #61646, .T. ) ;
#128394=FACE_OUTER_BOUND ( 'NONE', #11685, .T. ) ;
#128395=ORIENTED_EDGE ( 'NONE', *, *, #77926, .T. ) ;
#128396=ADVANCED_FACE ( 'NONE', ( #93243 ), #5182, .T. ) ;
#128397=ORIENTED_EDGE ( 'NONE', *, *, #105848, .F. ) ;
#128398=ORIENTED_EDGE ( 'NONE', *, *, #122718, .T. ) ;
#128399=EDGE_CURVE ( 'NONE', #116265, #123569, #61854, .T. ) ;
#128400=CIRCLE ( 'NONE', #101272, 0.06509327318403745899 ) ;
#128401=DIRECTION ( 'NONE',  ( 0.000000000000000000, 1.000000000000000000, 0.000000000000000000 ) ) ;
#128402=AXIS2_PLACEMENT_3D ( 'NONE', #101179, #22634, #62554 ) ;
#128403=CIRCLE ( 'NONE', #71955, 0.1000000000000002554 ) ;
#128404=ORIENTED_EDGE ( 'NONE', *, *, #53733, .F. ) ;
#128405=ORIENTED_EDGE ( 'NONE', *, *, #95683, .F. ) ;
#128406=DIRECTION ( 'NONE',  ( -0.000000000000000000, 1.000000000000000000, -0.000000000000000000 ) ) ;
#128407=EDGE_CURVE ( 'NONE', #129005, #52447, #60575, .T. ) ;
#128408=AXIS2_PLACEMENT_3D ( 'NONE', #77409, #85919, #17836 ) ;
#128409=CARTESIAN_POINT ( 'NONE',  ( 5.449999999999936229, 2.500000000000000000, -2.065063509461102065 ) ) ;
#128410=VECTOR ( 'NONE', #10708, 1000.000000000000000 ) ;
#128412=DIRECTION ( 'NONE',  ( -0.000000000000000000, -1.000000000000000000, -0.000000000000000000 ) ) ;
#128413=CARTESIAN_POINT ( 'NONE',  ( 12.29999999999990479, 12.50000000000000000, -4.048810130592463530 ) ) ;
#128414=ORIENTED_EDGE ( 'NONE', *, *, #66837, .F. ) ;
#128415=DIRECTION ( 'NONE',  ( 0.000000000000000000, -0.000000000000000000, 1.000000000000000000 ) ) ;
#128416=CIRCLE ( 'NONE', #126337, 0.1000000000000002554 ) ;
#128417=CIRCLE ( 'NONE', #88679, 0.06509327318403745899 ) ;
#128419=DIRECTION ( 'NONE',  ( 0.000000000000000000, 1.000000000000000000, 0.000000000000000000 ) ) ;
#128420=CIRCLE ( 'NONE', #48988, 0.09999999999999982514 ) ;
#128421=ORIENTED_EDGE ( 'NONE', *, *, #61078, .F. ) ;
#128422=CARTESIAN_POINT ( 'NONE',  ( 7.499999999999923617, 12.50000000000000000, 0.7579135962115869374 ) ) ;
#128423=ORIENTED_EDGE ( 'NONE', *, *, #16281, .T. ) ;
#128424=CONICAL_SURFACE ( 'NONE', #115864, 0.1000000000000002554, 0.003490658503988666988 ) ;
#128425=EDGE_CURVE ( 'NONE', #128215, #124558, #122292, .T. ) ;
#128426=EDGE_LOOP ( 'NONE', ( #113174, #81407 ) ) ;
#128427=CARTESIAN_POINT ( 'NONE',  ( -5.850000000000021849, 2.500000000000000000, -5.802370205355749988 ) ) ;
#128428=DIRECTION ( 'NONE',  ( -0.000000000000000000, 1.000000000000000000, -0.000000000000000000 ) ) ;
#128429=CARTESIAN_POINT ( 'NONE',  ( -2.300000000000033573, 12.50000000000000000, 4.741630453620009789 ) ) ;
#128430=DIRECTION ( 'NONE',  ( -0.000000000000000000, 1.000000000000000000, -0.000000000000000000 ) ) ;
#128431=LINE ( 'NONE', #98944, #74302 ) ;
#128432=ORIENTED_EDGE ( 'NONE', *, *, #29635, .F. ) ;
#128433=DIRECTION ( 'NONE',  ( 0.000000000000000000, 1.000000000000000000, 0.000000000000000000 ) ) ;
#128434=FACE_OUTER_BOUND ( 'NONE', #81518, .T. ) ;
#128435=FACE_OUTER_BOUND ( 'NONE', #127810, .T. ) ;
#128436=CARTESIAN_POINT ( 'NONE',  ( -8.750000000000005329, 12.50000000000000000, 5.737276932171707422 ) ) ;
#128437=AXIS2_PLACEMENT_3D ( 'NONE', #20269, #26013, #5701 ) ;
#128438=LINE ( 'NONE', #110693, #58196 ) ;
#128439=ORIENTED_EDGE ( 'NONE', *, *, #92153, .F. ) ;
#128440=EDGE_CURVE ( 'NONE', #48843, #63643, #121400, .T. ) ;
#128441=ORIENTED_EDGE ( 'NONE', *, *, #87055, .T. ) ;
#128442=CARTESIAN_POINT ( 'NONE',  ( 13.94999999999989271, 12.50000000000000000, -1.753560074763288679 ) ) ;
#128443=ORIENTED_EDGE ( 'NONE', *, *, #35200, .F. ) ;
#128444=CIRCLE ( 'NONE', #109553, 0.09999999999999982514 ) ;
#128445=CARTESIAN_POINT ( 'NONE',  ( 17.50000000000000000, -2.500000000000000000, 2.922290670089274567 ) ) ;
#128446=CARTESIAN_POINT ( 'NONE',  ( 9.599999999999914380, 12.50000000000000000, 3.572213422710607489 ) ) ;
#128447=AXIS2_PLACEMENT_3D ( 'NONE', #72605, #103995, #14303 ) ;
#128448=VERTEX_POINT ( 'NONE', #21931 ) ;
#128450=CARTESIAN_POINT ( 'NONE',  ( 13.94999999999989626, 2.500000000000000000, 2.411473670974873862 ) ) ;
#128451=EDGE_CURVE ( 'NONE', #79468, #61045, #90974, .T. ) ;
#128452=CARTESIAN_POINT ( 'NONE',  ( -10.85000000000000142, 12.50000000000000000, -1.537336459617583584 ) ) ;
#128453=CARTESIAN_POINT ( 'NONE',  ( 7.049999999999926992, 12.50000000000000000, 2.165063509461097713 ) ) ;
#128454=ORIENTED_EDGE ( 'NONE', *, *, #31536, .T. ) ;
#128455=AXIS2_PLACEMENT_3D ( 'NONE', #127945, #48755, #6216 ) ;
#128456=CARTESIAN_POINT ( 'NONE',  ( -13.14999999999999147, 2.500000000000000000, -2.411473670974875638 ) ) ;
#128457=ORIENTED_EDGE ( 'NONE', *, *, #5063, .F. ) ;
#128458=CARTESIAN_POINT ( 'NONE',  ( 26.61817589030699338, 2.722754549395931978, -4.358315860969328881 ) ) ;
#128459=CARTESIAN_POINT ( 'NONE',  ( 9.349999999999919709, 2.500000000000000000, -6.248780366869526759 ) ) ;
#128460=DIRECTION ( 'NONE',  ( 0.000000000000000000, 0.000000000000000000, -1.000000000000000000 ) ) ;
#128461=ORIENTED_EDGE ( 'NONE', *, *, #105863, .F. ) ;
#128462=AXIS2_PLACEMENT_3D ( 'NONE', #76623, #94309, #46501 ) ;
#128463=CARTESIAN_POINT ( 'NONE',  ( -1.650000000000034328, 2.500000000000000000, -7.288010851410854585 ) ) ;
#128464=AXIS2_PLACEMENT_3D ( 'NONE', #85179, #4656, #114008 ) ;
#128465=VERTEX_POINT ( 'NONE', #112235 ) ;
#128466=DIRECTION ( 'NONE',  ( -4.274815082592931898E-19, -0.9999939076577903929, -0.003490651415223739937 ) ) ;
#128468=DIRECTION ( 'NONE',  ( 0.000000000000000000, 1.000000000000000000, 0.000000000000000000 ) ) ;
#128469=VECTOR ( 'NONE', #45565, 1000.000000000000000 ) ;
#128470=ORIENTED_EDGE ( 'NONE', *, *, #46165, .T. ) ;
#128471=DIRECTION ( 'NONE',  ( 0.000000000000000000, 1.000000000000000000, 0.000000000000000000 ) ) ;
#128472=EDGE_CURVE ( 'NONE', #104829, #25799, #22589, .T. ) ;
#128473=FACE_OUTER_BOUND ( 'NONE', #58685, .T. ) ;
#128474=ORIENTED_EDGE ( 'NONE', *, *, #18242, .F. ) ;
#128475=CARTESIAN_POINT ( 'NONE',  ( 12.04999999999990479, 2.500000000000000000, -6.495190528383302464 ) ) ;
#128476=ORIENTED_EDGE ( 'NONE', *, *, #91738, .F. ) ;
#128477=LINE ( 'NONE', #55842, #53676 ) ;
#128478=EDGE_CURVE ( 'NONE', #19198, #113972, #30360, .T. ) ;
#128479=CIRCLE ( 'NONE', #103336, 0.06509327318403745899 ) ;
#128480=ORIENTED_EDGE ( 'NONE', *, *, #32835, .T. ) ;
#128481=FACE_OUTER_BOUND ( 'NONE', #79441, .T. ) ;
#128482=CARTESIAN_POINT ( 'NONE',  ( -1.650000000000035216, 12.50000000000000000, -1.472243186433550122 ) ) ;
#128483=AXIS2_PLACEMENT_3D ( 'NONE', #50177, #88793, #88113 ) ;
#128484=EDGE_CURVE ( 'NONE', #29292, #83964, #105639, .T. ) ;
#128485=AXIS2_PLACEMENT_3D ( 'NONE', #86134, #126076, #58648 ) ;
#128486=ORIENTED_EDGE ( 'NONE', *, *, #91360, .T. ) ;
#128487=ADVANCED_FACE ( 'NONE', ( #55878 ), #36903, .T. ) ;
#128488=ORIENTED_EDGE ( 'NONE', *, *, #112200, .T. ) ;
#128489=ADVANCED_FACE ( 'NONE', ( #106276 ), #19882, .T. ) ;
#128490=EDGE_CURVE ( 'NONE', #75076, #124980, #80524, .T. ) ;
#128491=DIRECTION ( 'NONE',  ( -4.274815082592931898E-19, -0.9999939076577903929, -0.003490651415223739937 ) ) ;
#128492=CARTESIAN_POINT ( 'NONE',  ( 3.749999999999942268, 2.500000000000000000, -5.902370205355750521 ) ) ;
#128493=ORIENTED_EDGE ( 'NONE', *, *, #2679, .F. ) ;
#128494=DIRECTION ( 'NONE',  ( 0.000000000000000000, 0.000000000000000000, 1.000000000000000000 ) ) ;
#128495=DIRECTION ( 'NONE',  ( 0.000000000000000000, 0.000000000000000000, 1.000000000000000000 ) ) ;
#128496=CIRCLE ( 'NONE', #113812, 0.06509327318403745899 ) ;
#128497=VECTOR ( 'NONE', #101622, 1000.000000000000000 ) ;
#128498=AXIS2_PLACEMENT_3D ( 'NONE', #23133, #33607, #73513 ) ;
#128499=FACE_OUTER_BOUND ( 'NONE', #128582, .T. ) ;
#128500=ADVANCED_FACE ( 'NONE', ( #75512 ), #125899, .T. ) ;
#128501=LINE ( 'NONE', #59759, #1247 ) ;
#128502=FACE_OUTER_BOUND ( 'NONE', #52095, .T. ) ;
#128503=AXIS2_PLACEMENT_3D ( 'NONE', #36668, #47126, #76578 ) ;
#128504=EDGE_CURVE ( 'NONE', #11437, #102844, #7429, .T. ) ;
#128506=CARTESIAN_POINT ( 'NONE',  ( -10.65000000000000213, 12.50000000000000000, 6.776507416713035248 ) ) ;
#128507=EDGE_CURVE ( 'NONE', #110767, #18837, #88923, .T. ) ;
#128509=AXIS2_PLACEMENT_3D ( 'NONE', #29242, #88789, #46949 ) ;
#128510=CIRCLE ( 'NONE', #109713, 0.1000000000000000472 ) ;
#128511=ADVANCED_FACE ( 'NONE', ( #95170 ), #47157, .T. ) ;
#128512=ORIENTED_EDGE ( 'NONE', *, *, #120509, .T. ) ;
#128513=ORIENTED_EDGE ( 'NONE', *, *, #54147, .T. ) ;
#128514=ORIENTED_EDGE ( 'NONE', *, *, #34396, .F. ) ;
#128516=FACE_OUTER_BOUND ( 'NONE', #46545, .T. ) ;
#128517=CARTESIAN_POINT ( 'NONE',  ( 11.24999999999994493, 2.500000000000000000, -2.165063509461101710 ) ) ;
#128518=AXIS2_PLACEMENT_3D ( 'NONE', #58694, #31187, #28595 ) ;
#128519=DIRECTION ( 'NONE',  ( 0.000000000000000000, 0.000000000000000000, 1.000000000000000000 ) ) ;
#128520=ORIENTED_EDGE ( 'NONE', *, *, #111281, .T. ) ;
#128521=FACE_BOUND ( 'NONE', #11779, .T. ) ;
#128522=ORIENTED_EDGE ( 'NONE', *, *, #21663, .T. ) ;
#128523=EDGE_CURVE ( 'NONE', #100830, #18875, #116092, .T. ) ;
#128524=CARTESIAN_POINT ( 'NONE',  ( 9.149999999999916866, 2.500000000000000000, 7.188010851410848723 ) ) ;
#128525=DIRECTION ( 'NONE',  ( -0.000000000000000000, 1.000000000000000000, -0.000000000000000000 ) ) ;
#128526=CARTESIAN_POINT ( 'NONE',  ( -10.84999999999999964, 12.50000000000000000, 1.472243186433545459 ) ) ;
#128527=CARTESIAN_POINT ( 'NONE',  ( -8.150000000000014566, 2.500000000000000000, -6.841600689897073373 ) ) ;
#128528=FACE_OUTER_BOUND ( 'NONE', #19329, .T. ) ;
#128529=DIRECTION ( 'NONE',  ( 0.000000000000000000, -0.000000000000000000, 1.000000000000000000 ) ) ;
#128530=DIRECTION ( 'NONE',  ( 0.000000000000000000, 1.000000000000000000, 0.000000000000000000 ) ) ;
#128531=DIRECTION ( 'NONE',  ( 0.000000000000000000, 1.000000000000000000, 0.000000000000000000 ) ) ;
#128532=FACE_OUTER_BOUND ( 'NONE', #109107, .T. ) ;
#128533=VECTOR ( 'NONE', #24401, 1000.000000000000000 ) ;
#128534=DIRECTION ( 'NONE',  ( 0.000000000000000000, 0.000000000000000000, 1.000000000000000000 ) ) ;
#128535=ORIENTED_EDGE ( 'NONE', *, *, #81501, .T. ) ;
#128536=ORIENTED_EDGE ( 'NONE', *, *, #111624, .T. ) ;
#128537=VERTEX_POINT ( 'NONE', #14649 ) ;
#128538=ORIENTED_EDGE ( 'NONE', *, *, #94147, .F. ) ;
#128539=DIRECTION ( 'NONE',  ( 0.000000000000000000, -0.9999939076577903929, 0.003490651415223739937 ) ) ;
#128540=DIRECTION ( 'NONE',  ( -0.000000000000000000, 1.000000000000000000, -0.000000000000000000 ) ) ;
#128541=EDGE_LOOP ( 'NONE', ( #75432, #98630, #27824, #106390 ) ) ;
#128542=ORIENTED_EDGE ( 'NONE', *, *, #47318, .T. ) ;
#128543=EDGE_LOOP ( 'NONE', ( #61999, #64732 ) ) ;
#128545=AXIS2_PLACEMENT_3D ( 'NONE', #106427, #16731, #7571 ) ;
#128546=AXIS2_PLACEMENT_3D ( 'NONE', #115733, #96728, #7057 ) ;
#128547=CARTESIAN_POINT ( 'NONE',  ( 13.74999999999989875, 2.500000000000000000, 1.472243186433545459 ) ) ;
#128548=FACE_OUTER_BOUND ( 'NONE', #114032, .T. ) ;
#128549=CARTESIAN_POINT ( 'NONE',  ( -10.85000000000000142, 2.500000000000000000, -2.757883832488650100 ) ) ;
#128550=DIRECTION ( 'NONE',  ( 0.000000000000000000, 1.000000000000000000, 0.000000000000000000 ) ) ;
#128551=FACE_OUTER_BOUND ( 'NONE', #78533, .T. ) ;
#128552=LINE ( 'NONE', #19185, #63565 ) ;
#128553=ORIENTED_EDGE ( 'NONE', *, *, #102488, .T. ) ;
#128554=PLANE ( 'NONE',  #55942 ) ;
#128555=VERTEX_POINT ( 'NONE', #35612 ) ;
#128556=CIRCLE ( 'NONE', #983, 0.06509327318403745899 ) ;
#128557=EDGE_CURVE ( 'NONE', #110134, #51506, #3244, .T. ) ;
#128558=ORIENTED_EDGE ( 'NONE', *, *, #70904, .T. ) ;
#128559=EDGE_LOOP ( 'NONE', ( #80572, #122542, #117462, #63304 ) ) ;
#128560=CONICAL_SURFACE ( 'NONE', #88810, 0.1000000000000002554, 0.003490658503988666988 ) ;
#128561=EDGE_CURVE ( 'NONE', #868, #85577, #94513, .T. ) ;
#128562=FACE_OUTER_BOUND ( 'NONE', #10984, .T. ) ;
#128564=ORIENTED_EDGE ( 'NONE', *, *, #35271, .T. ) ;
#128565=CARTESIAN_POINT ( 'NONE',  ( 3.749999999999942268, 12.50000000000000000, -5.802370205355749988 ) ) ;
#128566=EDGE_CURVE ( 'NONE', #128537, #16422, #114059, .T. ) ;
#128567=DIRECTION ( 'NONE',  ( 0.000000000000000000, 1.000000000000000000, 0.000000000000000000 ) ) ;
#128568=AXIS2_PLACEMENT_3D ( 'NONE', #25246, #16708, #127350 ) ;
#128569=ADVANCED_FACE ( 'NONE', ( #4832 ), #25776, .T. ) ;
#128570=CARTESIAN_POINT ( 'NONE',  ( 3.299999999999944755, 12.50000000000000000, -4.330127018922201643 ) ) ;
#128571=AXIS2_PLACEMENT_3D ( 'NONE', #33674, #72319, #73578 ) ;
#128572=LINE ( 'NONE', #17933, #14839 ) ;
#128573=CARTESIAN_POINT ( 'NONE',  ( -6.650000000000015454, 12.50000000000000000, 7.122917578226811486 ) ) ;
#128575=AXIS2_PLACEMENT_3D ( 'NONE', #90623, #2899, #101742 ) ;
#128576=CARTESIAN_POINT ( 'NONE',  ( 13.74999999999993072, 2.500000000000000000, -2.265063509461101798 ) ) ;
#128577=ORIENTED_EDGE ( 'NONE', *, *, #12865, .T. ) ;
#128578=CARTESIAN_POINT ( 'NONE',  ( 16.56034315062901641, -0.8287392047036244991, 6.090234455234610600 ) ) ;
#128579=ORIENTED_EDGE ( 'NONE', *, *, #119181, .T. ) ;
#128580=DIRECTION ( 'NONE',  ( -0.000000000000000000, 1.000000000000000000, -0.000000000000000000 ) ) ;
#128581=FACE_OUTER_BOUND ( 'NONE', #58378, .T. ) ;
#128582=EDGE_LOOP ( 'NONE', ( #66541, #72841, #124338, #61079 ) ) ;
#128583=CARTESIAN_POINT ( 'NONE',  ( 9.149999999999920419, 2.500000000000000000, 1.472243186433545459 ) ) ;
#128584=DIRECTION ( 'NONE',  ( 0.000000000000000000, 0.000000000000000000, 1.000000000000000000 ) ) ;
#128585=VERTEX_POINT ( 'NONE', #74889 ) ;
#128586=VECTOR ( 'NONE', #2997, 1000.000000000000000 ) ;
#128587=FACE_OUTER_BOUND ( 'NONE', #67488, .T. ) ;
#128588=EDGE_LOOP ( 'NONE', ( #2052, #108065, #10818, #2446 ) ) ;
#128589=AXIS2_PLACEMENT_3D ( 'NONE', #36766, #37407, #5344 ) ;
#128590=EDGE_LOOP ( 'NONE', ( #60305, #91895 ) ) ;
#128591=DIRECTION ( 'NONE',  ( 0.000000000000000000, 1.000000000000000000, 0.000000000000000000 ) ) ;
#128592=CARTESIAN_POINT ( 'NONE',  ( 12.09999999999990550, 12.50000000000000000, 3.637306695894644726 ) ) ;
#128594=DIRECTION ( 'NONE',  ( 0.000000000000000000, 0.000000000000000000, -1.000000000000000000 ) ) ;
#128595=EDGE_CURVE ( 'NONE', #83042, #70566, #78478, .T. ) ;
#128596=AXIS2_PLACEMENT_3D ( 'NONE', #91506, #102604, #32621 ) ;
#128597=DIRECTION ( 'NONE',  ( -0.000000000000000000, 1.000000000000000000, -0.000000000000000000 ) ) ;
#128598=CONICAL_SURFACE ( 'NONE', #57471, 0.09999999999999999167, 0.003490658503988666988 ) ;
#128599=ORIENTED_EDGE ( 'NONE', *, *, #61256, .F. ) ;
#128600=AXIS2_PLACEMENT_3D ( 'NONE', #54630, #65089, #4235 ) ;
#128601=CARTESIAN_POINT ( 'NONE',  ( -10.60000000000000142, 2.500000000000000000, 3.983716857408420964 ) ) ;
#128602=AXIS2_PLACEMENT_3D ( 'NONE', #118267, #28615, #46301 ) ;
#128603=EDGE_LOOP ( 'NONE', ( #70471, #23873 ) ) ;
#128604=CIRCLE ( 'NONE', #120170, 0.1000000000000000472 ) ;
#128605=DIRECTION ( 'NONE',  ( 0.000000000000000000, 1.000000000000000000, 0.000000000000000000 ) ) ;
#128606=CARTESIAN_POINT ( 'NONE',  ( 1.649999999999951505, 2.500000000000000000, -1.472243186433550122 ) ) ;
#128607=AXIS2_PLACEMENT_3D ( 'NONE', #121399, #31740, #90651 ) ;
#128608=ORIENTED_EDGE ( 'NONE', *, *, #81033, .F. ) ;
#128609=CONICAL_SURFACE ( 'NONE', #17752, 0.1000000000000002554, 0.003490658503988666988 ) ;
#128610=ADVANCED_FACE ( 'NONE', ( #104963 ), #109855, .T. ) ;
#128611=DIRECTION ( 'NONE',  ( -0.000000000000000000, -1.000000000000000000, -0.000000000000000000 ) ) ;
#128612=LINE ( 'NONE', #116813, #38520 ) ;
#128613=CARTESIAN_POINT ( 'NONE',  ( 6.049999999999935874, 12.50000000000000000, -6.776507416713039689 ) ) ;
#128614=ADVANCED_FACE ( 'NONE', ( #65702 ), #19968, .T. ) ;
#128615=CARTESIAN_POINT ( 'NONE',  ( 10.39999999999991509, 2.500000000000000000, -0.5928203230275542746 ) ) ;
#128616=DIRECTION ( 'NONE',  ( 0.000000000000000000, -0.000000000000000000, 1.000000000000000000 ) ) ;
#128618=DIRECTION ( 'NONE',  ( 0.000000000000000000, 1.000000000000000000, 0.000000000000000000 ) ) ;
#128619=DIRECTION ( 'NONE',  ( -0.000000000000000000, -1.000000000000000000, -0.000000000000000000 ) ) ;
#128620=DIRECTION ( 'NONE',  ( 0.000000000000000000, -0.000000000000000000, 1.000000000000000000 ) ) ;
#128621=EDGE_CURVE ( 'NONE', #59948, #112383, #108840, .T. ) ;
#128622=CIRCLE ( 'NONE', #40792, 0.06509327318403745899 ) ;
#128623=EDGE_LOOP ( 'NONE', ( #83903, #62938 ) ) ;
#128624=FACE_OUTER_BOUND ( 'NONE', #1756, .T. ) ;
#128625=ORIENTED_EDGE ( 'NONE', *, *, #104454, .F. ) ;
#128626=ORIENTED_EDGE ( 'NONE', *, *, #122795, .T. ) ;
#128627=DIRECTION ( 'NONE',  ( 0.000000000000000000, -0.9999939076577903929, 0.003490651415223739937 ) ) ;
#128628=CONICAL_SURFACE ( 'NONE', #15712, 0.1000000000000002554, 0.003490658503988666988 ) ;
#128629=ORIENTED_EDGE ( 'NONE', *, *, #93567, .F. ) ;
#128630=PLANE ( 'NONE',  #59092 ) ;
#128631=CARTESIAN_POINT ( 'NONE',  ( -8.550000000000007816, 2.500000000000000000, 6.048780366869520364 ) ) ;
#128632=AXIS2_PLACEMENT_3D ( 'NONE', #1625, #42216, #51406 ) ;
#128633=AXIS2_PLACEMENT_3D ( 'NONE', #54717, #67094, #85481 ) ;
#128634=ORIENTED_EDGE ( 'NONE', *, *, #18494, .F. ) ;
#128635=CARTESIAN_POINT ( 'NONE',  ( 13.94999999999989271, 12.50000000000000000, -1.883746621131363597 ) ) ;
#128636=CARTESIAN_POINT ( 'NONE',  ( -14.99999999999998401, 2.500000000000000000, 0.6928203230275518099 ) ) ;
#128637=ORIENTED_EDGE ( 'NONE', *, *, #128930, .T. ) ;
#128639=DIRECTION ( 'NONE',  ( 0.000000000000000000, 1.000000000000000000, 0.000000000000000000 ) ) ;
#128640=ORIENTED_EDGE ( 'NONE', *, *, #96867, .F. ) ;
#128641=CIRCLE ( 'NONE', #90964, 0.06509327318403745899 ) ;
#128642=EDGE_CURVE ( 'NONE', #104109, #124072, #42978, .T. ) ;
#128643=ORIENTED_EDGE ( 'NONE', *, *, #20621, .T. ) ;
#128644=VECTOR ( 'NONE', #65360, 1000.000000000000000 ) ;
#128645=EDGE_LOOP ( 'NONE', ( #36634, #81636 ) ) ;
#128646=CARTESIAN_POINT ( 'NONE',  ( -6.850000000000017408, 2.500000000000000000, -2.511473670974877948 ) ) ;
#128647=CARTESIAN_POINT ( 'NONE',  ( -0.4000000000000396572, 2.500000000000000000, 4.330127018922196314 ) ) ;
#128648=CARTESIAN_POINT ( 'NONE',  ( 4.399999999999940847, 2.500000000000000000, -4.576537180435977348 ) ) ;
#128649=EDGE_CURVE ( 'NONE', #58785, #11040, #29020, .T. ) ;
#128650=FACE_BOUND ( 'NONE', #4634, .T. ) ;
#128651=VERTEX_POINT ( 'NONE', #57827 ) ;
#128652=EDGE_CURVE ( 'NONE', #81351, #47988, #47361, .T. ) ;
#128653=EDGE_CURVE ( 'NONE', #43124, #8732, #5277, .T. ) ;
#128654=CARTESIAN_POINT ( 'NONE',  ( 7.499999999999961808, 12.50000000000000000, 4.395220292106234439 ) ) ;
#128655=CARTESIAN_POINT ( 'NONE',  ( 3.299999999999942979, 2.500000000000000000, 4.330127018922196314 ) ) ;
#128656=ORIENTED_EDGE ( 'NONE', *, *, #75293, .T. ) ;
#128657=LINE ( 'NONE', #78901, #61226 ) ;
#128658=CARTESIAN_POINT ( 'NONE',  ( -11.25000000000000178, 2.500000000000000000, -5.802370205355746435 ) ) ;
#128659=AXIS2_PLACEMENT_3D ( 'NONE', #56521, #65037, #26435 ) ;
#128660=EDGE_CURVE ( 'NONE', #113932, #50402, #70148, .T. ) ;
#128661=FACE_OUTER_BOUND ( 'NONE', #49472, .T. ) ;
#128662=CARTESIAN_POINT ( 'NONE',  ( 3.299999999999944755, 12.50000000000000000, -2.385244779468109755E-15 ) ) ;
#128663=CARTESIAN_POINT ( 'NONE',  ( 8.099999999999923261, 2.500000000000000000, 3.983716857408420076 ) ) ;
#128664=EDGE_CURVE ( 'NONE', #128960, #73467, #34656, .T. ) ;
#128665=CARTESIAN_POINT ( 'NONE',  ( 1.899999999999951283, 2.500000000000000000, -4.776537180435977525 ) ) ;
#128666=CARTESIAN_POINT ( 'NONE',  ( -1.900000000000034550, 2.500000000000000000, 4.576537180435972019 ) ) ;
#128667=EDGE_CURVE ( 'NONE', #29752, #12644, #119306, .T. ) ;
#128668=VERTEX_POINT ( 'NONE', #78770 ) ;
#128669=ORIENTED_EDGE ( 'NONE', *, *, #78524, .T. ) ;
#128670=EDGE_LOOP ( 'NONE', ( #68526, #34813 ) ) ;
#128671=CIRCLE ( 'NONE', #82689, 0.06509327318403745899 ) ;
#128672=VERTEX_POINT ( 'NONE', #38185 ) ;
#128673=ORIENTED_EDGE ( 'NONE', *, *, #45469, .T. ) ;
#128674=CARTESIAN_POINT ( 'NONE',  ( 9.999999999999952038, 2.500000000000000000, 0.09999999999999772959 ) ) ;
#128675=FACE_OUTER_BOUND ( 'NONE', #79021, .T. ) ;
#128676=ORIENTED_EDGE ( 'NONE', *, *, #58885, .T. ) ;
#128677=ADVANCED_FACE ( 'NONE', ( #168 ), #28287, .T. ) ;
#128678=FACE_BOUND ( 'NONE', #5864, .T. ) ;
#128679=AXIS2_PLACEMENT_3D ( 'NONE', #104062, #74601, #3921 ) ;
#128680=ADVANCED_FACE ( 'NONE', ( #118022 ), #101440, .T. ) ;
#128681=FACE_OUTER_BOUND ( 'NONE', #47861, .T. ) ;
#128682=CONICAL_SURFACE ( 'NONE', #53350, 0.1000000000000000472, 0.003490658503988666988 ) ;
#128683=DIRECTION ( 'NONE',  ( 0.000000000000000000, 0.000000000000000000, 1.000000000000000000 ) ) ;
#128684=AXIS2_PLACEMENT_3D ( 'NONE', #72239, #11365, #93166 ) ;
#128685=DIRECTION ( 'NONE',  ( 0.000000000000000000, 0.000000000000000000, 1.000000000000000000 ) ) ;
#128686=DIRECTION ( 'NONE',  ( 0.000000000000000000, 0.000000000000000000, 1.000000000000000000 ) ) ;
#128687=CARTESIAN_POINT ( 'NONE',  ( 12.49999999999993605, 2.500000000000000000, 0.09999999999999772959 ) ) ;
#128688=ORIENTED_EDGE ( 'NONE', *, *, #31536, .F. ) ;
#128689=AXIS2_PLACEMENT_3D ( 'NONE', #44034, #93138, #54480 ) ;
#128690=ORIENTED_EDGE ( 'NONE', *, *, #34551, .F. ) ;
#128691=AXIS2_PLACEMENT_3D ( 'NONE', #12261, #41757, #63305 ) ;
#128692=AXIS2_PLACEMENT_3D ( 'NONE', #85241, #6019, #34877 ) ;
#128693=VERTEX_POINT ( 'NONE', #57170 ) ;
#128694=ORIENTED_EDGE ( 'NONE', *, *, #92352, .F. ) ;
#128695=CARTESIAN_POINT ( 'NONE',  ( 12.04999999999990479, 2.500000000000000000, -6.395190528383301931 ) ) ;
#128696=VECTOR ( 'NONE', #84133, 1000.000000000000000 ) ;
#128697=CARTESIAN_POINT ( 'NONE',  ( 6.049999999999935874, 12.50000000000000000, -6.841600689897077814 ) ) ;
#128698=DIRECTION ( 'NONE',  ( 0.000000000000000000, 0.000000000000000000, 1.000000000000000000 ) ) ;
#128699=ORIENTED_EDGE ( 'NONE', *, *, #103761, .T. ) ;
#128700=DIRECTION ( 'NONE',  ( 0.000000000000000000, 0.000000000000000000, 1.000000000000000000 ) ) ;
#128701=AXIS2_PLACEMENT_3D ( 'NONE', #31180, #129390, #1049 ) ;
#128702=CIRCLE ( 'NONE', #88961, 0.06509327318403745899 ) ;
#128703=FACE_OUTER_BOUND ( 'NONE', #16746, .T. ) ;
#128704=AXIS2_PLACEMENT_3D ( 'NONE', #62371, #22456, #14523 ) ;
#128705=DIRECTION ( 'NONE',  ( 0.000000000000000000, 0.000000000000000000, 1.000000000000000000 ) ) ;
#128707=DIRECTION ( 'NONE',  ( -0.000000000000000000, -1.000000000000000000, -0.000000000000000000 ) ) ;
#128708=DIRECTION ( 'NONE',  ( -4.274815082592931898E-19, -0.9999939076577903929, -0.003490651415223739937 ) ) ;
#128710=DIRECTION ( 'NONE',  ( 0.000000000000000000, 0.000000000000000000, 1.000000000000000000 ) ) ;
#128711=ORIENTED_EDGE ( 'NONE', *, *, #98321, .F. ) ;
#128712=FACE_OUTER_BOUND ( 'NONE', #23204, .T. ) ;
#128713=ORIENTED_EDGE ( 'NONE', *, *, #100673, .T. ) ;
#128714=EDGE_CURVE ( 'NONE', #14057, #127872, #95182, .T. ) ;
#128715=VERTEX_POINT ( 'NONE', #19839 ) ;
#128716=PLANE ( 'NONE',  #109516 ) ;
#128717=EDGE_CURVE ( 'NONE', #4956, #117143, #116102, .T. ) ;
#128718=CARTESIAN_POINT ( 'NONE',  ( 2.899999999999944844, 12.50000000000000000, 5.088040615133786027 ) ) ;
#128719=DIRECTION ( 'NONE',  ( 0.000000000000000000, 0.000000000000000000, 1.000000000000000000 ) ) ;
#128720=CIRCLE ( 'NONE', #107754, 0.06509327318403741736 ) ;
#128721=EDGE_LOOP ( 'NONE', ( #3826, #34119, #12043, #31449 ) ) ;
#128723=CARTESIAN_POINT ( 'NONE',  ( -7.500000000000016875, 2.500000000000000000, 0.6928203230275494784 ) ) ;
#128724=DIRECTION ( 'NONE',  ( -0.000000000000000000, 1.000000000000000000, -0.000000000000000000 ) ) ;
#128725=DIRECTION ( 'NONE',  ( 0.000000000000000000, -0.9999939076577903929, 0.003490651415223739937 ) ) ;
#128726=ORIENTED_EDGE ( 'NONE', *, *, #60362, .T. ) ;
#128727=CARTESIAN_POINT ( 'NONE',  ( 4.199999999999938005, 2.500000000000000000, 4.230127018922196669 ) ) ;
#128728=CIRCLE ( 'NONE', #38840, 0.1000000000000000472 ) ;
#128729=ORIENTED_EDGE ( 'NONE', *, *, #15820, .F. ) ;
#128730=DIRECTION ( 'NONE',  ( -0.000000000000000000, 1.000000000000000000, -0.000000000000000000 ) ) ;
#128731=CIRCLE ( 'NONE', #20045, 0.06509327318403745899 ) ;
#128732=ORIENTED_EDGE ( 'NONE', *, *, #21194, .T. ) ;
#128733=CARTESIAN_POINT ( 'NONE',  ( -9.350000000000006750, 12.50000000000000000, 2.511473670974873507 ) ) ;
#128734=CARTESIAN_POINT ( 'NONE',  ( 0.3999999999999568345, 12.50000000000000000, -3.702399969078687292 ) ) ;
#128735=DIRECTION ( 'NONE',  ( 0.000000000000000000, 0.000000000000000000, 1.000000000000000000 ) ) ;
#128736=CARTESIAN_POINT ( 'NONE',  ( -9.600000000000008527, 2.500000000000000000, -5.022947341949749678 ) ) ;
#128737=EDGE_LOOP ( 'NONE', ( #27019, #9034 ) ) ;
#128738=AXIS2_PLACEMENT_3D ( 'NONE', #56308, #127004, #77252 ) ;
#128739=DIRECTION ( 'NONE',  ( -0.000000000000000000, 1.000000000000000000, -0.000000000000000000 ) ) ;
#128740=CIRCLE ( 'NONE', #72285, 0.1000000000000000472 ) ;
#128741=VERTEX_POINT ( 'NONE', #129169 ) ;
#128742=ORIENTED_EDGE ( 'NONE', *, *, #4797, .F. ) ;
#128743=DIRECTION ( 'NONE',  ( 0.000000000000000000, 0.000000000000000000, 1.000000000000000000 ) ) ;
#128744=FACE_OUTER_BOUND ( 'NONE', #97070, .T. ) ;
#128745=FACE_OUTER_BOUND ( 'NONE', #58875, .T. ) ;
#128746=CARTESIAN_POINT ( 'NONE',  ( 11.89999999999990798, 2.500000000000000000, 4.776537180435972196 ) ) ;
#128747=CARTESIAN_POINT ( 'NONE',  ( -6.250000000000019540, 2.500000000000000000, -7.088010851410853519 ) ) ;
#128748=DIRECTION ( 'NONE',  ( 0.000000000000000000, 0.000000000000000000, 1.000000000000000000 ) ) ;
#128749=EDGE_CURVE ( 'NONE', #118039, #36428, #80613, .T. ) ;
#128750=CIRCLE ( 'NONE', #53418, 0.09999999999999982514 ) ;
#128751=CONICAL_SURFACE ( 'NONE', #95273, 0.1000000000000002554, 0.003490658503988666988 ) ;
#128752=FACE_OUTER_BOUND ( 'NONE', #114335, .T. ) ;
#128753=CARTESIAN_POINT ( 'NONE',  ( -0.2000000000000412836, 12.50000000000000000, 4.676537180435972552 ) ) ;
#128754=CARTESIAN_POINT ( 'NONE',  ( 1.849999999999949019, 2.500000000000000000, 6.841600689897072485 ) ) ;
#128755=ADVANCED_FACE ( 'NONE', ( #109499 ), #45015, .T. ) ;
#128756=VERTEX_POINT ( 'NONE', #40119 ) ;
#128757=DIRECTION ( 'NONE',  ( 0.000000000000000000, -0.000000000000000000, 1.000000000000000000 ) ) ;
#128758=EDGE_CURVE ( 'NONE', #8842, #45024, #1178, .T. ) ;
#128759=DIRECTION ( 'NONE',  ( 0.000000000000000000, 1.000000000000000000, 0.000000000000000000 ) ) ;
#128760=DIRECTION ( 'NONE',  ( 0.000000000000000000, 0.000000000000000000, -1.000000000000000000 ) ) ;
#128761=EDGE_CURVE ( 'NONE', #92171, #57040, #91065, .T. ) ;
#128762=CARTESIAN_POINT ( 'NONE',  ( 2.099999999999947686, 2.500000000000000000, 5.022947341949748790 ) ) ;
#128763=DIRECTION ( 'NONE',  ( 0.000000000000000000, 0.000000000000000000, 1.000000000000000000 ) ) ;
#128764=EDGE_LOOP ( 'NONE', ( #44471, #119545, #71517, #33322 ) ) ;
#128765=CARTESIAN_POINT ( 'NONE',  ( -11.05000000000000071, 12.50000000000000000, -6.776507416713037912 ) ) ;
#128766=AXIS2_PLACEMENT_3D ( 'NONE', #83429, #123342, #107570 ) ;
#128767=CIRCLE ( 'NONE', #93244, 0.1000000000000002554 ) ;
#128768=CARTESIAN_POINT ( 'NONE',  ( 6.249999999999930722, 12.50000000000000000, 7.122917578226811486 ) ) ;
#128769=CARTESIAN_POINT ( 'NONE',  ( -2.900000000000029221, 2.500000000000000000, -0.7928203230275542301 ) ) ;
#128770=ORIENTED_EDGE ( 'NONE', *, *, #27216, .T. ) ;
#128771=ADVANCED_FACE ( 'NONE', ( #10011 ), #36702, .T. ) ;
#128772=ORIENTED_EDGE ( 'NONE', *, *, #45253, .T. ) ;
#128773=CARTESIAN_POINT ( 'NONE',  ( 14.34999999999989662, 2.500000000000000000, 1.818653347947321475 ) ) ;
#128774=ORIENTED_EDGE ( 'NONE', *, *, #102033, .T. ) ;
#128775=ORIENTED_EDGE ( 'NONE', *, *, #22980, .T. ) ;
#128776=ORIENTED_EDGE ( 'NONE', *, *, #75812, .T. ) ;
#128777=DIRECTION ( 'NONE',  ( -0.000000000000000000, -1.000000000000000000, -0.000000000000000000 ) ) ;
#128778=AXIS2_PLACEMENT_3D ( 'NONE', #60513, #263, #69662 ) ;
#128779=DIRECTION ( 'NONE',  ( -0.000000000000000000, -1.000000000000000000, -0.000000000000000000 ) ) ;
#128780=DIRECTION ( 'NONE',  ( 0.000000000000000000, -0.000000000000000000, 1.000000000000000000 ) ) ;
#128781=AXIS2_PLACEMENT_3D ( 'NONE', #81410, #109571, #51314 ) ;
#128782=DIRECTION ( 'NONE',  ( 0.000000000000000000, -0.9999939076577903929, 0.003490651415223739937 ) ) ;
#128783=AXIS2_PLACEMENT_3D ( 'NONE', #89061, #87750, #22 ) ;
#128784=ORIENTED_EDGE ( 'NONE', *, *, #50168, .T. ) ;
#128785=AXIS2_PLACEMENT_3D ( 'NONE', #16455, #96309, #86496 ) ;
#128786=DIRECTION ( 'NONE',  ( 0.000000000000000000, 1.000000000000000000, 0.000000000000000000 ) ) ;
#128787=AXIS2_PLACEMENT_3D ( 'NONE', #87666, #9120, #37938 ) ;
#128788=VERTEX_POINT ( 'NONE', #97100 ) ;
#128789=CARTESIAN_POINT ( 'NONE',  ( -2.500000000000032863, 12.50000000000000000, 5.022947341949748790 ) ) ;
#128790=CARTESIAN_POINT ( 'NONE',  ( 18.37149739118984471, -2.540880845001673105, -2.596776292463405245 ) ) ;
#128791=CARTESIAN_POINT ( 'NONE',  ( 16.58100817950494843, 2.557139044001653261, 6.067820687733449958 ) ) ;
#128792=DIRECTION ( 'NONE',  ( 0.000000000000000000, 0.000000000000000000, -1.000000000000000000 ) ) ;
#128793=CARTESIAN_POINT ( 'NONE',  ( 3.549999999999943867, 2.500000000000000000, -1.818653347947326138 ) ) ;
#128794=VERTEX_POINT ( 'NONE', #30959 ) ;
#128797=EDGE_LOOP ( 'NONE', ( #51414, #25883 ) ) ;
#128798=ORIENTED_EDGE ( 'NONE', *, *, #72385, .F. ) ;
#128799=ORIENTED_EDGE ( 'NONE', *, *, #63764, .T. ) ;
#128800=DIRECTION ( 'NONE',  ( 0.000000000000000000, 1.000000000000000000, 0.000000000000000000 ) ) ;
#128801=DIRECTION ( 'NONE',  ( 0.000000000000000000, 0.000000000000000000, -1.000000000000000000 ) ) ;
#128802=CARTESIAN_POINT ( 'NONE',  ( -7.500000000000015099, 2.500000000000000000, -4.922947341949753586 ) ) ;
#128803=EDGE_CURVE ( 'NONE', #39135, #384, #32893, .T. ) ;
#128804=FACE_BOUND ( 'NONE', #12895, .T. ) ;
#128805=DIRECTION ( 'NONE',  ( 0.000000000000000000, 1.000000000000000000, 0.000000000000000000 ) ) ;
#128806=AXIS2_PLACEMENT_3D ( 'NONE', #16890, #104651, #35298 ) ;
#128807=DIRECTION ( 'NONE',  ( -0.000000000000000000, -1.000000000000000000, -0.000000000000000000 ) ) ;
#128808=ADVANCED_FACE ( 'NONE', ( #30317 ), #118158, .T. ) ;
#128809=DIRECTION ( 'NONE',  ( 0.000000000000000000, 0.000000000000000000, -1.000000000000000000 ) ) ;
#128810=DIRECTION ( 'NONE',  ( 0.000000000000000000, 1.000000000000000000, 0.000000000000000000 ) ) ;
#128811=EDGE_CURVE ( 'NONE', #28513, #17110, #110777, .T. ) ;
#128812=CARTESIAN_POINT ( 'NONE',  ( 10.84999999999990905, 12.50000000000000000, -6.560283801567339701 ) ) ;
#128813=EDGE_CURVE ( 'NONE', #127159, #109486, #62346, .T. ) ;
#128814=CONICAL_SURFACE ( 'NONE', #1330, 0.1000000000000002554, 0.003490658503988666988 ) ;
#128815=DIRECTION ( 'NONE',  ( -0.000000000000000000, 1.000000000000000000, -0.000000000000000000 ) ) ;
#128816=ADVANCED_FACE ( 'NONE', ( #21111 ), #70224, .T. ) ;
#128817=DIRECTION ( 'NONE',  ( -0.000000000000000000, 1.000000000000000000, -0.000000000000000000 ) ) ;
#128818=AXIS2_PLACEMENT_3D ( 'NONE', #74868, #114774, #25111 ) ;
#128819=ADVANCED_FACE ( 'NONE', ( #92432 ), #41425, .T. ) ;
#128820=AXIS2_PLACEMENT_3D ( 'NONE', #3546, #43487, #81472 ) ;
#128821=CARTESIAN_POINT ( 'NONE',  ( 4.149999999999941735, 12.50000000000000000, -1.472243186433550122 ) ) ;
#128822=CONICAL_SURFACE ( 'NONE', #80680, 0.1000000000000002554, 0.003490658503988666988 ) ;
#128823=ADVANCED_FACE ( 'NONE', ( #120609 ), #82768, .T. ) ;
#128824=ORIENTED_EDGE ( 'NONE', *, *, #4, .T. ) ;
#128825=ORIENTED_EDGE ( 'NONE', *, *, #67455, .T. ) ;
#128826=ORIENTED_EDGE ( 'NONE', *, *, #87183, .F. ) ;
#128827=ORIENTED_EDGE ( 'NONE', *, *, #103073, .T. ) ;
#128828=DIRECTION ( 'NONE',  ( 0.000000000000000000, 0.000000000000000000, 1.000000000000000000 ) ) ;
#128829=DIRECTION ( 'NONE',  ( -0.000000000000000000, 1.000000000000000000, -0.000000000000000000 ) ) ;
#128830=FACE_BOUND ( 'NONE', #47527, .T. ) ;
#128831=ADVANCED_FACE ( 'NONE', ( #91794 ), #9594, .T. ) ;
#128832=AXIS2_PLACEMENT_3D ( 'NONE', #48285, #88175, #78407 ) ;
#128833=CARTESIAN_POINT ( 'NONE',  ( 10.19999999999991225, 2.500000000000000000, -4.776537180435978414 ) ) ;
#128834=CIRCLE ( 'NONE', #95355, 0.1000000000000000472 ) ;
#128835=VECTOR ( 'NONE', #10623, 1000.000000000000000 ) ;
#128836=EDGE_LOOP ( 'NONE', ( #62443, #82864 ) ) ;
#128837=DIRECTION ( 'NONE',  ( 0.000000000000000000, 0.000000000000000000, 1.000000000000000000 ) ) ;
#128838=DIRECTION ( 'NONE',  ( -4.274815082592931898E-19, -0.9999939076577903929, -0.003490651415223739937 ) ) ;
#128839=CARTESIAN_POINT ( 'NONE',  ( -0.6500000000000394351, 12.50000000000000000, 6.841600689897072485 ) ) ;
#128840=DIRECTION ( 'NONE',  ( 0.000000000000000000, 0.000000000000000000, -1.000000000000000000 ) ) ;
#128841=DIRECTION ( 'NONE',  ( 0.000000000000000000, -0.000000000000000000, 1.000000000000000000 ) ) ;
#128842=VERTEX_POINT ( 'NONE', #121254 ) ;
#128843=CARTESIAN_POINT ( 'NONE',  ( 6.849999999999927702, 2.500000000000000000, 2.511473670974873507 ) ) ;
#128844=VERTEX_POINT ( 'NONE', #11289 ) ;
#128845=ORIENTED_EDGE ( 'NONE', *, *, #73747, .F. ) ;
#128846=CARTESIAN_POINT ( 'NONE',  ( 9.599999999999914380, 2.500000000000000000, -5.022947341949754119 ) ) ;
#128848=ORIENTED_EDGE ( 'NONE', *, *, #28583, .F. ) ;
#128849=DIRECTION ( 'NONE',  ( 0.000000000000000000, 0.000000000000000000, -1.000000000000000000 ) ) ;
#128850=CARTESIAN_POINT ( 'NONE',  ( 2.099999999999949463, 12.50000000000000000, 0.7579135962115869374 ) ) ;
#128851=EDGE_LOOP ( 'NONE', ( #10842, #101063 ) ) ;
#128852=DIRECTION ( 'NONE',  ( -0.000000000000000000, -1.000000000000000000, -0.000000000000000000 ) ) ;
#128853=ORIENTED_EDGE ( 'NONE', *, *, #53719, .T. ) ;
#128854=DIRECTION ( 'NONE',  ( 0.000000000000000000, 1.000000000000000000, 0.000000000000000000 ) ) ;
#128856=DIRECTION ( 'NONE',  ( 0.000000000000000000, -0.000000000000000000, 1.000000000000000000 ) ) ;
#128857=FACE_BOUND ( 'NONE', #106640, .T. ) ;
#128858=AXIS2_PLACEMENT_3D ( 'NONE', #13871, #4051, #44001 ) ;
#128860=EDGE_CURVE ( 'NONE', #16485, #59989, #28381, .T. ) ;
#128862=EDGE_LOOP ( 'NONE', ( #13314, #121822 ) ) ;
#128863=LINE ( 'NONE', #21452, #65930 ) ;
#128864=DIRECTION ( 'NONE',  ( 0.000000000000000000, 0.000000000000000000, 1.000000000000000000 ) ) ;
#128865=FACE_OUTER_BOUND ( 'NONE', #46862, .T. ) ;
#128866=CARTESIAN_POINT ( 'NONE',  ( -8.300000000000009592, 2.500000000000000000, 4.430127018922196847 ) ) ;
#128867=DIRECTION ( 'NONE',  ( 0.000000000000000000, 1.000000000000000000, 0.000000000000000000 ) ) ;
#128868=EDGE_LOOP ( 'NONE', ( #120402, #96814, #12455, #10062 ) ) ;
#128869=AXIS2_PLACEMENT_3D ( 'NONE', #2040, #60966, #121179 ) ;
#128870=CIRCLE ( 'NONE', #61948, 0.06509327318403745899 ) ;
#128871=VERTEX_POINT ( 'NONE', #1466 ) ;
#128872=EDGE_CURVE ( 'NONE', #2945, #88713, #116182, .T. ) ;
#128873=ORIENTED_EDGE ( 'NONE', *, *, #5355, .F. ) ;
#128874=CARTESIAN_POINT ( 'NONE',  ( 8.149999999999920419, 12.50000000000000000, 6.148780366869520897 ) ) ;
#128875=DIRECTION ( 'NONE',  ( 0.000000000000000000, 0.000000000000000000, 1.000000000000000000 ) ) ;
#128876=DIRECTION ( 'NONE',  ( -0.000000000000000000, 1.000000000000000000, -0.000000000000000000 ) ) ;
#128877=EDGE_LOOP ( 'NONE', ( #138, #99904, #64537, #119606 ) ) ;
#128878=VERTEX_POINT ( 'NONE', #71501 ) ;
#128879=ORIENTED_EDGE ( 'NONE', *, *, #112106, .F. ) ;
#128880=CARTESIAN_POINT ( 'NONE',  ( -12.69999999999999218, 12.50000000000000000, -4.676537180435975216 ) ) ;
#128881=CONICAL_SURFACE ( 'NONE', #116221, 0.1000000000000000472, 0.003490658503988666988 ) ;
#128882=DIRECTION ( 'NONE',  ( 0.000000000000000000, 0.000000000000000000, 1.000000000000000000 ) ) ;
#128883=AXIS2_PLACEMENT_3D ( 'NONE', #86335, #106629, #77176 ) ;
#128884=DIRECTION ( 'NONE',  ( 0.000000000000000000, 0.000000000000000000, -1.000000000000000000 ) ) ;
#128885=DIRECTION ( 'NONE',  ( 0.000000000000000000, 0.000000000000000000, 1.000000000000000000 ) ) ;
#128886=DIRECTION ( 'NONE',  ( -0.000000000000000000, 1.000000000000000000, -0.000000000000000000 ) ) ;
#128887=CARTESIAN_POINT ( 'NONE',  ( 1.649999999999951505, 2.500000000000000000, -2.857883832488653741 ) ) ;
#128888=DIRECTION ( 'NONE',  ( 0.000000000000000000, 0.000000000000000000, 1.000000000000000000 ) ) ;
#128889=LINE ( 'NONE', #18255, #129415 ) ;
#128890=ORIENTED_EDGE ( 'NONE', *, *, #48222, .T. ) ;
#128891=ORIENTED_EDGE ( 'NONE', *, *, #87419, .T. ) ;
#128892=DIRECTION ( 'NONE',  ( -0.000000000000000000, 1.000000000000000000, -0.000000000000000000 ) ) ;
#128893=DIRECTION ( 'NONE',  ( -0.000000000000000000, 1.000000000000000000, -0.000000000000000000 ) ) ;
#128894=ORIENTED_EDGE ( 'NONE', *, *, #79004, .T. ) ;
#128895=VERTEX_POINT ( 'NONE', #42055 ) ;
#128896=CARTESIAN_POINT ( 'NONE',  ( -9.150000000000005684, 12.50000000000000000, 5.802370205355744659 ) ) ;
#128897=DIRECTION ( 'NONE',  ( 0.000000000000000000, 1.000000000000000000, 0.000000000000000000 ) ) ;
#128898=AXIS2_PLACEMENT_3D ( 'NONE', #129496, #79721, #90159 ) ;
#128899=CARTESIAN_POINT ( 'NONE',  ( 3.749999999999940492, 2.500000000000000000, 2.957883832488649389 ) ) ;
#128900=DIRECTION ( 'NONE',  ( 0.000000000000000000, 0.000000000000000000, -1.000000000000000000 ) ) ;
#128901=EDGE_CURVE ( 'NONE', #106998, #24838, #111414, .T. ) ;
#128902=DIRECTION ( 'NONE',  ( 0.000000000000000000, -0.9999939076577903929, 0.003490651415223739937 ) ) ;
#128903=CIRCLE ( 'NONE', #53656, 0.1000000000000000472 ) ;
#128904=LINE ( 'NONE', #120991, #69907 ) ;
#128905=DIRECTION ( 'NONE',  ( 0.000000000000000000, 0.000000000000000000, 1.000000000000000000 ) ) ;
#128906=CONICAL_SURFACE ( 'NONE', #59862, 0.1000000000000002554, 0.003490658503988666988 ) ;
#128907=CIRCLE ( 'NONE', #72449, 0.1000000000000002554 ) ;
#128908=AXIS2_PLACEMENT_3D ( 'NONE', #58463, #19820, #28350 ) ;
#128909=CARTESIAN_POINT ( 'NONE',  ( -0.4000000000000401013, 12.50000000000000000, -3.637306695894650055 ) ) ;
#128910=EDGE_CURVE ( 'NONE', #129385, #98295, #61705, .T. ) ;
#128911=EDGE_LOOP ( 'NONE', ( #98741, #20546 ) ) ;
#128912=AXIS2_PLACEMENT_3D ( 'NONE', #129100, #66910, #77394 ) ;
#128913=ORIENTED_EDGE ( 'NONE', *, *, #78247, .F. ) ;
#128914=ADVANCED_FACE ( 'NONE', ( #51878 ), #76496, .T. ) ;
#128915=ORIENTED_EDGE ( 'NONE', *, *, #100524, .F. ) ;
#128916=ORIENTED_EDGE ( 'NONE', *, *, #66593, .T. ) ;
#128917=EDGE_CURVE ( 'NONE', #54589, #24400, #101535, .T. ) ;
#128918=DIRECTION ( 'NONE',  ( -4.274815082592931898E-19, -0.9999939076577903929, -0.003490651415223739937 ) ) ;
#128919=FACE_OUTER_BOUND ( 'NONE', #63410, .T. ) ;
#128920=CIRCLE ( 'NONE', #93388, 0.06509327318403745899 ) ;
#128921=ORIENTED_EDGE ( 'NONE', *, *, #101024, .T. ) ;
#128922=DIRECTION ( 'NONE',  ( 0.000000000000000000, 0.000000000000000000, -1.000000000000000000 ) ) ;
#128923=CARTESIAN_POINT ( 'NONE',  ( 0.6499999999999561684, 2.500000000000000000, 1.718653347947321386 ) ) ;
#128924=CIRCLE ( 'NONE', #97499, 0.1000000000000000472 ) ;
#128925=CONICAL_SURFACE ( 'NONE', #78738, 0.1000000000000002554, 0.003490658503988666988 ) ;
#128926=ADVANCED_FACE ( 'NONE', ( #43353 ), #5333, .T. ) ;
#128927=CARTESIAN_POINT ( 'NONE',  ( -6.850000000000013856, 12.50000000000000000, 6.148780366869520897 ) ) ;
#128928=CARTESIAN_POINT ( 'NONE',  ( -12.09999999999999609, 2.500000000000000000, -4.230127018922199333 ) ) ;
#128929=ORIENTED_EDGE ( 'NONE', *, *, #7205, .T. ) ;
#128930=EDGE_CURVE ( 'NONE', #70003, #527, #103689, .T. ) ;
#128931=DIRECTION ( 'NONE',  ( 0.000000000000000000, 1.000000000000000000, 0.000000000000000000 ) ) ;
#128932=CARTESIAN_POINT ( 'NONE',  ( 4.999999999999973355, 2.500000000000000000, -4.330127018922201643 ) ) ;
#128933=ORIENTED_EDGE ( 'NONE', *, *, #24452, .T. ) ;
#128934=EDGE_LOOP ( 'NONE', ( #43152, #48373 ) ) ;
#128935=ORIENTED_EDGE ( 'NONE', *, *, #230, .F. ) ;
#128936=VERTEX_POINT ( 'NONE', #23699 ) ;
#128937=CARTESIAN_POINT ( 'NONE',  ( -8.150000000000014566, 2.500000000000000000, -6.048780366869521252 ) ) ;
#128938=PLANE ( 'NONE',  #32018 ) ;
#128939=PLANE ( 'NONE',  #62865 ) ;
#128940=ORIENTED_EDGE ( 'NONE', *, *, #42036, .F. ) ;
#128941=FACE_OUTER_BOUND ( 'NONE', #9615, .T. ) ;
#128942=CARTESIAN_POINT ( 'NONE',  ( 6.049999999999930544, 2.500000000000000000, 2.511473670974873507 ) ) ;
#128943=FACE_OUTER_BOUND ( 'NONE', #30216, .T. ) ;
#128944=DIRECTION ( 'NONE',  ( -0.000000000000000000, 1.000000000000000000, -0.000000000000000000 ) ) ;
#128945=ORIENTED_EDGE ( 'NONE', *, *, #96960, .F. ) ;
#128946=AXIS2_PLACEMENT_3D ( 'NONE', #11787, #51093, #72017 ) ;
#128947=DIRECTION ( 'NONE',  ( 0.000000000000000000, -0.9999939076577903929, 0.003490651415223739937 ) ) ;
#128948=AXIS2_PLACEMENT_3D ( 'NONE', #107322, #57593, #97504 ) ;
#128949=ORIENTED_EDGE ( 'NONE', *, *, #126600, .F. ) ;
#128950=ORIENTED_EDGE ( 'NONE', *, *, #85932, .F. ) ;
#128951=DIRECTION ( 'NONE',  ( 0.000000000000000000, -0.000000000000000000, 1.000000000000000000 ) ) ;
#128952=DIRECTION ( 'NONE',  ( 0.000000000000000000, 1.000000000000000000, 0.000000000000000000 ) ) ;
#128953=FACE_BOUND ( 'NONE', #15829, .T. ) ;
#128954=DIRECTION ( 'NONE',  ( -4.274815082592931898E-19, -0.9999939076577903929, -0.003490651415223739937 ) ) ;
#128955=FACE_OUTER_BOUND ( 'NONE', #114194, .T. ) ;
#128956=AXIS2_PLACEMENT_3D ( 'NONE', #116506, #87043, #126985 ) ;
#128957=CONICAL_SURFACE ( 'NONE', #66227, 0.09999999999999982514, 0.003490658503988666988 ) ;
#128958=CARTESIAN_POINT ( 'NONE',  ( 8.349999999999923261, 12.50000000000000000, -7.188010851410854052 ) ) ;
#128959=EDGE_CURVE ( 'NONE', #96953, #83685, #83273, .T. ) ;
#128960=VERTEX_POINT ( 'NONE', #15137 ) ;
#128961=EDGE_CURVE ( 'NONE', #18164, #11592, #66019, .T. ) ;
#128962=DIRECTION ( 'NONE',  ( 0.000000000000000000, 0.000000000000000000, 1.000000000000000000 ) ) ;
#128963=DIRECTION ( 'NONE',  ( 0.000000000000000000, 0.000000000000000000, -1.000000000000000000 ) ) ;
#128964=AXIS2_PLACEMENT_3D ( 'NONE', #93733, #94361, #115943 ) ;
#128965=DIRECTION ( 'NONE',  ( 0.000000000000000000, -0.9999939076577903929, 0.003490651415223739937 ) ) ;
#128966=EDGE_CURVE ( 'NONE', #116101, #58516, #123198, .T. ) ;
#128968=VERTEX_POINT ( 'NONE', #93728 ) ;
#128969=CIRCLE ( 'NONE', #16044, 0.06509327318403745899 ) ;
#128970=CIRCLE ( 'NONE', #57854, 0.06509327318403745899 ) ;
#128971=ADVANCED_FACE ( 'NONE', ( #94358 ), #128751, .T. ) ;
#128972=DIRECTION ( 'NONE',  ( -4.274815082592931898E-19, -0.9999939076577903929, -0.003490651415223739937 ) ) ;
#128973=AXIS2_PLACEMENT_3D ( 'NONE', #61847, #42868, #82779 ) ;
#128974=CARTESIAN_POINT ( 'NONE',  ( -8.150000000000012790, 2.500000000000000000, -2.511473670974877948 ) ) ;
#128975=EDGE_CURVE ( 'NONE', #12077, #79693, #65550, .T. ) ;
#128976=VERTEX_POINT ( 'NONE', #5969 ) ;
#128977=VERTEX_POINT ( 'NONE', #124480 ) ;
#128978=CARTESIAN_POINT ( 'NONE',  ( -11.89999999999999503, 2.500000000000000000, 4.676537180435972552 ) ) ;
#128980=FACE_BOUND ( 'NONE', #22373, .T. ) ;
#128981=DIRECTION ( 'NONE',  ( 0.000000000000000000, 1.000000000000000000, 0.000000000000000000 ) ) ;
#128982=EDGE_CURVE ( 'NONE', #92222, #72461, #41014, .T. ) ;
#128983=EDGE_CURVE ( 'NONE', #30750, #8254, #15840, .T. ) ;
#128984=DIRECTION ( 'NONE',  ( 0.000000000000000000, -0.9999939076577903929, 0.003490651415223739937 ) ) ;
#128985=ORIENTED_EDGE ( 'NONE', *, *, #127668, .T. ) ;
#128986=FACE_OUTER_BOUND ( 'NONE', #82402, .T. ) ;
#128988=AXIS2_PLACEMENT_3D ( 'NONE', #78939, #69746, #8237 ) ;
#128989=AXIS2_PLACEMENT_3D ( 'NONE', #117861, #128367, #9860 ) ;
#128990=EDGE_CURVE ( 'NONE', #30644, #3252, #32608, .T. ) ;
#128991=VERTEX_POINT ( 'NONE', #85823 ) ;
#128992=DIRECTION ( 'NONE',  ( 0.000000000000000000, -0.9999939076577903929, 0.003490651415223739937 ) ) ;
#128994=FACE_OUTER_BOUND ( 'NONE', #28264, .T. ) ;
#128995=CONICAL_SURFACE ( 'NONE', #66263, 0.1000000000000000472, 0.003490658503988666988 ) ;
#128996=CARTESIAN_POINT ( 'NONE',  ( 6.649999999999930189, 2.500000000000000000, 5.802370205355744659 ) ) ;
#128997=LINE ( 'NONE', #39329, #78191 ) ;
#128998=AXIS2_PLACEMENT_3D ( 'NONE', #37061, #78280, #18688 ) ;
#128999=EDGE_LOOP ( 'NONE', ( #78827, #8125 ) ) ;
#129000=CIRCLE ( 'NONE', #13945, 0.06509327318403745899 ) ;
#129002=DIRECTION ( 'NONE',  ( 0.000000000000000000, -0.000000000000000000, 1.000000000000000000 ) ) ;
#129003=DIRECTION ( 'NONE',  ( 0.000000000000000000, 1.000000000000000000, 0.000000000000000000 ) ) ;
#129004=CARTESIAN_POINT ( 'NONE',  ( 7.299999999999926104, 2.500000000000000000, -4.083716857408426826 ) ) ;
#129005=VERTEX_POINT ( 'NONE', #105482 ) ;
#129006=ORIENTED_EDGE ( 'NONE', *, *, #94480, .F. ) ;
#129007=AXIS2_PLACEMENT_3D ( 'NONE', #25463, #106612, #86319 ) ;
#129008=CARTESIAN_POINT ( 'NONE',  ( 16.98389447545206821, 2.499999999999373390, 5.627887033857345678 ) ) ;
#129009=AXIS2_PLACEMENT_3D ( 'NONE', #43316, #83235, #73392 ) ;
#129010=ORIENTED_EDGE ( 'NONE', *, *, #120544, .T. ) ;
#129011=PLANE ( 'NONE',  #91102 ) ;
#129012=DIRECTION ( 'NONE',  ( 0.000000000000000000, -0.000000000000000000, 1.000000000000000000 ) ) ;
#129013=CARTESIAN_POINT ( 'NONE',  ( 1.049999999999952083, 12.50000000000000000, 6.841600689897072485 ) ) ;
#129014=CIRCLE ( 'NONE', #82933, 0.1000000000000002554 ) ;
#129015=CONICAL_SURFACE ( 'NONE', #11901, 0.09999999999999982514, 0.003490658503988666988 ) ;
#129016=CARTESIAN_POINT ( 'NONE',  ( -8.150000000000014566, 2.500000000000000000, -6.741600689897072840 ) ) ;
#129017=ORIENTED_EDGE ( 'NONE', *, *, #65670, .F. ) ;
#129019=CARTESIAN_POINT ( 'NONE',  ( -3.950000000000026379, 2.500000000000000000, 6.941600689897073018 ) ) ;
#129020=DIRECTION ( 'NONE',  ( 0.000000000000000000, -0.9999939076577903929, 0.003490651415223739937 ) ) ;
#129022=DIRECTION ( 'NONE',  ( 0.000000000000000000, 1.000000000000000000, 0.000000000000000000 ) ) ;
#129023=DIRECTION ( 'NONE',  ( -0.000000000000000000, -1.000000000000000000, -0.000000000000000000 ) ) ;
#129024=ORIENTED_EDGE ( 'NONE', *, *, #79971, .T. ) ;
#129025=ADVANCED_FACE ( 'NONE', ( #95021 ), #74439, .T. ) ;
#129026=ORIENTED_EDGE ( 'NONE', *, *, #95623, .F. ) ;
#129027=DIRECTION ( 'NONE',  ( -0.000000000000000000, 1.000000000000000000, -0.000000000000000000 ) ) ;
#129029=DIRECTION ( 'NONE',  ( -4.274815082592931898E-19, -0.9999939076577903929, -0.003490651415223739937 ) ) ;
#129031=ORIENTED_EDGE ( 'NONE', *, *, #109950, .F. ) ;
#129032=ORIENTED_EDGE ( 'NONE', *, *, #63273, .F. ) ;
#129033=CONICAL_SURFACE ( 'NONE', #36973, 0.1000000000000002554, 0.003490658503988666988 ) ;
#129034=CARTESIAN_POINT ( 'NONE',  ( 11.24999999999994316, 12.50000000000000000, 2.165063509461097713 ) ) ;
#129035=DIRECTION ( 'NONE',  ( 0.000000000000000000, 1.000000000000000000, 0.000000000000000000 ) ) ;
#129036=DIRECTION ( 'NONE',  ( -0.000000000000000000, 1.000000000000000000, -0.000000000000000000 ) ) ;
#129037=FACE_OUTER_BOUND ( 'NONE', #32838, .T. ) ;
#129038=LINE ( 'NONE', #89727, #81452 ) ;
#129040=DIRECTION ( 'NONE',  ( -0.000000000000000000, -1.000000000000000000, -0.000000000000000000 ) ) ;
#129041=CARTESIAN_POINT ( 'NONE',  ( 3.549999999999943867, 2.500000000000000000, -6.148780366869526226 ) ) ;
#129042=ORIENTED_EDGE ( 'NONE', *, *, #63273, .T. ) ;
#129043=VECTOR ( 'NONE', #68619, 1000.000000000000000 ) ;
#129044=ORIENTED_EDGE ( 'NONE', *, *, #58939, .F. ) ;
#129045=CIRCLE ( 'NONE', #108078, 0.06509327318403745899 ) ;
#129046=DIRECTION ( 'NONE',  ( -0.000000000000000000, 1.000000000000000000, -0.000000000000000000 ) ) ;
#129047=EDGE_LOOP ( 'NONE', ( #52585, #16791 ) ) ;
#129048=ORIENTED_EDGE ( 'NONE', *, *, #73101, .T. ) ;
#129049=DIRECTION ( 'NONE',  ( 0.000000000000000000, 1.000000000000000000, 0.000000000000000000 ) ) ;
#129050=CIRCLE ( 'NONE', #3633, 0.06509327318403745899 ) ;
#129052=CARTESIAN_POINT ( 'NONE',  ( -1.250000000000001110, 2.500000000000000000, -6.495190528383302464 ) ) ;
#129053=DIRECTION ( 'NONE',  ( 0.000000000000000000, 0.000000000000000000, 1.000000000000000000 ) ) ;
#129054=CARTESIAN_POINT ( 'NONE',  ( 9.799999999999913669, 2.500000000000000000, 4.776537180435972196 ) ) ;
#129055=FACE_OUTER_BOUND ( 'NONE', #84531, .T. ) ;
#129056=ORIENTED_EDGE ( 'NONE', *, *, #45277, .T. ) ;
#129057=AXIS2_PLACEMENT_3D ( 'NONE', #68513, #67868, #105390 ) ;
#129058=VECTOR ( 'NONE', #70664, 1000.000000000000000 ) ;
#129059=VERTEX_POINT ( 'NONE', #15795 ) ;
#129060=CARTESIAN_POINT ( 'NONE',  ( 8.349999999999923261, 12.50000000000000000, -7.253104124594891289 ) ) ;
#129061=AXIS2_PLACEMENT_3D ( 'NONE', #157, #29638, #19827 ) ;
#129062=EDGE_CURVE ( 'NONE', #27571, #942, #3329, .T. ) ;
#129063=ORIENTED_EDGE ( 'NONE', *, *, #59570, .T. ) ;
#129064=DIRECTION ( 'NONE',  ( 0.000000000000000000, 0.000000000000000000, 1.000000000000000000 ) ) ;
#129065=VERTEX_POINT ( 'NONE', #114643 ) ;
#129066=ADVANCED_FACE ( 'NONE', ( #66187 ), #49327, .T. ) ;
#129067=ORIENTED_EDGE ( 'NONE', *, *, #68678, .F. ) ;
#129068=ADVANCED_FACE ( 'NONE', ( #106121 ), #14499, .T. ) ;
#129069=FACE_OUTER_BOUND ( 'NONE', #73189, .T. ) ;
#129070=FACE_OUTER_BOUND ( 'NONE', #28331, .T. ) ;
#129071=AXIS2_PLACEMENT_3D ( 'NONE', #31747, #101775, #13380 ) ;
#129072=DIRECTION ( 'NONE',  ( -0.000000000000000000, 1.000000000000000000, -0.000000000000000000 ) ) ;
#129073=CARTESIAN_POINT ( 'NONE',  ( -14.34999999999998543, 2.500000000000000000, -1.918653347947323784 ) ) ;
#129074=EDGE_CURVE ( 'NONE', #68346, #115529, #26327, .T. ) ;
#129075=DIRECTION ( 'NONE',  ( 0.000000000000000000, 0.000000000000000000, 1.000000000000000000 ) ) ;
#129077=ORIENTED_EDGE ( 'NONE', *, *, #96681, .F. ) ;
#129078=DIRECTION ( 'NONE',  ( 0.000000000000000000, 0.000000000000000000, 1.000000000000000000 ) ) ;
#129079=CARTESIAN_POINT ( 'NONE',  ( 8.349999999999919709, 12.50000000000000000, 7.122917578226811486 ) ) ;
#129080=EDGE_CURVE ( 'NONE', #40491, #66554, #39342, .T. ) ;
#129081=DIRECTION ( 'NONE',  ( 0.000000000000000000, 1.000000000000000000, 0.000000000000000000 ) ) ;
#129082=EDGE_CURVE ( 'NONE', #46559, #47762, #59798, .T. ) ;
#129083=EDGE_CURVE ( 'NONE', #98725, #83167, #57720, .T. ) ;
#129084=CARTESIAN_POINT ( 'NONE',  ( 12.89999999999990088, 2.500000000000000000, -4.230127018922201998 ) ) ;
#129085=CONICAL_SURFACE ( 'NONE', #72624, 0.09999999999999982514, 0.003490658503988666988 ) ;
#129086=CIRCLE ( 'NONE', #9924, 0.06509327318403745899 ) ;
#129087=DIRECTION ( 'NONE',  ( 0.000000000000000000, -0.9999939076577903929, 0.003490651415223739937 ) ) ;
#129088=ORIENTED_EDGE ( 'NONE', *, *, #33726, .T. ) ;
#129089=AXIS2_PLACEMENT_3D ( 'NONE', #29743, #69012, #17983 ) ;
#129090=ORIENTED_EDGE ( 'NONE', *, *, #69895, .T. ) ;
#129091=FACE_OUTER_BOUND ( 'NONE', #84712, .T. ) ;
#129092=EDGE_CURVE ( 'NONE', #27226, #41372, #84795, .T. ) ;
#129093=AXIS2_PLACEMENT_3D ( 'NONE', #53961, #23864, #103046 ) ;
#129094=ORIENTED_EDGE ( 'NONE', *, *, #50634, .F. ) ;
#129095=CARTESIAN_POINT ( 'NONE',  ( 17.50000000000000000, -2.499999999999960476, 3.093175630837758483 ) ) ;
#129097=AXIS2_PLACEMENT_3D ( 'NONE', #77234, #37956, #27468 ) ;
#129098=ORIENTED_EDGE ( 'NONE', *, *, #24648, .F. ) ;
#129099=DIRECTION ( 'NONE',  ( 0.000000000000000000, 0.000000000000000000, -1.000000000000000000 ) ) ;
#129100=CARTESIAN_POINT ( 'NONE',  ( -11.24999999999999822, 2.500000000000000000, 1.472243186433545459 ) ) ;
#129101=AXIS2_PLACEMENT_3D ( 'NONE', #18233, #118370, #69925 ) ;
#129102=PLANE ( 'NONE',  #98393 ) ;
#129103=DIRECTION ( 'NONE',  ( 0.000000000000000000, 1.000000000000000000, 0.000000000000000000 ) ) ;
#129104=VERTEX_POINT ( 'NONE', #57004 ) ;
#129105=CIRCLE ( 'NONE', #74695, 0.1000000000000002554 ) ;
#129106=CIRCLE ( 'NONE', #24527, 0.06509327318403745899 ) ;
#129107=LINE ( 'NONE', #39440, #35260 ) ;
#129108=ORIENTED_EDGE ( 'NONE', *, *, #108538, .F. ) ;
#129109=CARTESIAN_POINT ( 'NONE',  ( 8.349999999999919709, 2.500000000000000000, 6.495190528383297135 ) ) ;
#129110=DIRECTION ( 'NONE',  ( -0.000000000000000000, -1.000000000000000000, -0.000000000000000000 ) ) ;
#129111=CARTESIAN_POINT ( 'NONE',  ( 2.699999999999947331, 2.500000000000000000, -4.576537180435978236 ) ) ;
#129112=ORIENTED_EDGE ( 'NONE', *, *, #24278, .T. ) ;
#129113=DIRECTION ( 'NONE',  ( -0.000000000000000000, -1.000000000000000000, -0.000000000000000000 ) ) ;
#129114=ORIENTED_EDGE ( 'NONE', *, *, #92293, .F. ) ;
#129115=EDGE_CURVE ( 'NONE', #32550, #29908, #22546, .T. ) ;
#129116=DIRECTION ( 'NONE',  ( 0.000000000000000000, 1.000000000000000000, 0.000000000000000000 ) ) ;
#129117=CARTESIAN_POINT ( 'NONE',  ( -0.6000000000000388356, 2.500000000000000000, 4.676537180435972552 ) ) ;
#129118=CIRCLE ( 'NONE', #47533, 0.06509327318403745899 ) ;
#129119=CARTESIAN_POINT ( 'NONE',  ( 4.149999999999939959, 12.50000000000000000, -2.165063509461101710 ) ) ;
#129120=ADVANCED_FACE ( 'NONE', ( #96936 ), #68492, .T. ) ;
#129121=ORIENTED_EDGE ( 'NONE', *, *, #78405, .T. ) ;
#129122=DIRECTION ( 'NONE',  ( 0.000000000000000000, 0.000000000000000000, 1.000000000000000000 ) ) ;
#129123=EDGE_CURVE ( 'NONE', #2269, #118223, #16240, .T. ) ;
#129124=CARTESIAN_POINT ( 'NONE',  ( 9.399999999999915090, 12.50000000000000000, -3.983716857408426293 ) ) ;
#129125=ORIENTED_EDGE ( 'NONE', *, *, #125520, .F. ) ;
#129126=FACE_OUTER_BOUND ( 'NONE', #44189, .T. ) ;
#129127=ADVANCED_FACE ( 'NONE', ( #37394 ), #126993, .T. ) ;
#129128=ORIENTED_EDGE ( 'NONE', *, *, #122856, .T. ) ;
#129129=CARTESIAN_POINT ( 'NONE',  ( -11.25000000000000000, 2.500000000000000000, -7.188010851410850499 ) ) ;
#129130=EDGE_CURVE ( 'NONE', #11303, #72411, #77304, .T. ) ;
#129132=ADVANCED_FACE ( 'NONE', ( #120929 ), #111087, .T. ) ;
#129133=ADVANCED_FACE ( 'NONE', ( #27538 ), #116513, .T. ) ;
#129136=DIRECTION ( 'NONE',  ( 0.000000000000000000, 0.000000000000000000, 1.000000000000000000 ) ) ;
#129137=VERTEX_POINT ( 'NONE', #76665 ) ;
#129138=ORIENTED_EDGE ( 'NONE', *, *, #113835, .F. ) ;
#129139=CARTESIAN_POINT ( 'NONE',  ( -10.84999999999999964, 2.500000000000000000, 1.472243186433545459 ) ) ;
#129140=DIRECTION ( 'NONE',  ( -0.000000000000000000, -1.000000000000000000, -0.000000000000000000 ) ) ;
#129141=ORIENTED_EDGE ( 'NONE', *, *, #111965, .F. ) ;
#129143=AXIS2_PLACEMENT_3D ( 'NONE', #106321, #58529, #15987 ) ;
#129146=CIRCLE ( 'NONE', #72692, 0.06509327318403745899 ) ;
#129147=DIRECTION ( 'NONE',  ( 0.000000000000000000, -0.000000000000000000, 1.000000000000000000 ) ) ;
#129148=DIRECTION ( 'NONE',  ( 0.000000000000000000, 0.000000000000000000, 1.000000000000000000 ) ) ;
#129149=FACE_OUTER_BOUND ( 'NONE', #103391, .T. ) ;
#129150=DIRECTION ( 'NONE',  ( 0.000000000000000000, 0.000000000000000000, -1.000000000000000000 ) ) ;
#129151=CARTESIAN_POINT ( 'NONE',  ( -12.49999999999999289, 12.50000000000000000, 5.022947341949748790 ) ) ;
#129152=VECTOR ( 'NONE', #17040, 1000.000000000000000 ) ;
#129154=ORIENTED_EDGE ( 'NONE', *, *, #15380, .F. ) ;
#129155=ORIENTED_EDGE ( 'NONE', *, *, #73708, .F. ) ;
#129156=ORIENTED_EDGE ( 'NONE', *, *, #76603, .T. ) ;
#129157=DIRECTION ( 'NONE',  ( 0.000000000000000000, 1.000000000000000000, 0.000000000000000000 ) ) ;
#129158=CARTESIAN_POINT ( 'NONE',  ( -8.550000000000013145, 12.50000000000000000, 2.576566944158910744 ) ) ;
#129159=CIRCLE ( 'NONE', #116602, 0.06509327318403745899 ) ;
#129160=CARTESIAN_POINT ( 'NONE',  ( -1.850000000000033840, 12.50000000000000000, 6.841600689897072485 ) ) ;
#129161=VERTEX_POINT ( 'NONE', #86472 ) ;
#129162=FACE_BOUND ( 'NONE', #26915, .T. ) ;
#129163=ORIENTED_EDGE ( 'NONE', *, *, #99674, .T. ) ;
#129164=EDGE_CURVE ( 'NONE', #6313, #89626, #93540, .T. ) ;
#129165=DIRECTION ( 'NONE',  ( 0.000000000000000000, 0.000000000000000000, 1.000000000000000000 ) ) ;
#129166=LINE ( 'NONE', #100953, #12248 ) ;
#129167=CARTESIAN_POINT ( 'NONE',  ( -8.350000000000012079, 12.50000000000000000, 2.792790559304612064 ) ) ;
#129168=CIRCLE ( 'NONE', #104096, 0.06509327318403745899 ) ;
#129169=CARTESIAN_POINT ( 'NONE',  ( -8.950000000000009948, 2.500000000000000000, -1.718653347947326049 ) ) ;
#129170=CARTESIAN_POINT ( 'NONE',  ( -13.34999999999999076, 2.500000000000000000, 2.757883832488653209 ) ) ;
#129171=CONICAL_SURFACE ( 'NONE', #30867, 0.09999999999999982514, 0.003490658503988666988 ) ;
#129172=DIRECTION ( 'NONE',  ( -4.274815082592931898E-19, -0.9999939076577903929, -0.003490651415223739937 ) ) ;
#129173=ORIENTED_EDGE ( 'NONE', *, *, #93672, .T. ) ;
#129174=CARTESIAN_POINT ( 'NONE',  ( 10.79999999999991012, 2.500000000000000000, 4.330127018922196314 ) ) ;
#129175=CARTESIAN_POINT ( 'NONE',  ( 1.449999999999952216, 2.500000000000000000, 1.918653347947321564 ) ) ;
#129176=CONICAL_SURFACE ( 'NONE', #47588, 0.09999999999999982514, 0.003490658503988666988 ) ;
#129177=CIRCLE ( 'NONE', #85316, 0.06509327318403745899 ) ;
#129178=CARTESIAN_POINT ( 'NONE',  ( -6.700000000000019718, 12.50000000000000000, -4.330127018922201643 ) ) ;
#129179=ORIENTED_EDGE ( 'NONE', *, *, #79714, .F. ) ;
#129180=VECTOR ( 'NONE', #32353, 1000.000000000000000 ) ;
#129181=ORIENTED_EDGE ( 'NONE', *, *, #52377, .T. ) ;
#129182=EDGE_CURVE ( 'NONE', #92915, #104745, #108046, .T. ) ;
#129183=EDGE_LOOP ( 'NONE', ( #107860, #21727, #15972, #63592 ) ) ;
#129184=VERTEX_POINT ( 'NONE', #116573 ) ;
#129185=FACE_OUTER_BOUND ( 'NONE', #46274, .T. ) ;
#129186=CARTESIAN_POINT ( 'NONE',  ( -5.600000000000020073, 2.500000000000000000, 4.576537180435972019 ) ) ;
#129188=ORIENTED_EDGE ( 'NONE', *, *, #107753, .T. ) ;
#129189=EDGE_LOOP ( 'NONE', ( #65343, #115600, #113816, #121964 ) ) ;
#129190=CONICAL_SURFACE ( 'NONE', #120742, 0.09999999999999982514, 0.003490658503988666988 ) ;
#129191=VERTEX_POINT ( 'NONE', #49155 ) ;
#129192=CARTESIAN_POINT ( 'NONE',  ( 5.799999999999934985, 12.50000000000000000, -4.265033745738164406 ) ) ;
#129193=AXIS2_PLACEMENT_3D ( 'NONE', #38467, #65314, #96707 ) ;
#129194=FACE_OUTER_BOUND ( 'NONE', #106079, .T. ) ;
#129195=DIRECTION ( 'NONE',  ( 0.000000000000000000, 0.000000000000000000, 1.000000000000000000 ) ) ;
#129196=PLANE ( 'NONE',  #56346 ) ;
#129201=ADVANCED_FACE ( 'NONE', ( #18376 ), #58327, .T. ) ;
#129202=EDGE_LOOP ( 'NONE', ( #83003, #111553 ) ) ;
#129203=CARTESIAN_POINT ( 'NONE',  ( -8.350000000000012079, 2.500000000000000000, 1.572243186433545548 ) ) ;
#129204=VERTEX_POINT ( 'NONE', #68765 ) ;
#129205=VECTOR ( 'NONE', #33570, 1000.000000000000000 ) ;
#129206=VECTOR ( 'NONE', #27633, 1000.000000000000000 ) ;
#129207=ORIENTED_EDGE ( 'NONE', *, *, #70681, .T. ) ;
#129208=VERTEX_POINT ( 'NONE', #108695 ) ;
#129209=FACE_OUTER_BOUND ( 'NONE', #61513, .T. ) ;
#129210=ORIENTED_EDGE ( 'NONE', *, *, #65421, .T. ) ;
#129211=ORIENTED_EDGE ( 'NONE', *, *, #66525, .F. ) ;
#129213=CARTESIAN_POINT ( 'NONE',  ( 4.599999999999936584, 12.50000000000000000, 4.330127018922196314 ) ) ;
#129214=DIRECTION ( 'NONE',  ( 0.000000000000000000, 0.000000000000000000, 1.000000000000000000 ) ) ;
#129215=DIRECTION ( 'NONE',  ( 0.000000000000000000, 1.000000000000000000, 0.000000000000000000 ) ) ;
#129216=DIRECTION ( 'NONE',  ( -0.000000000000000000, -1.000000000000000000, -0.000000000000000000 ) ) ;
#129217=ORIENTED_EDGE ( 'NONE', *, *, #38369, .F. ) ;
#129218=CARTESIAN_POINT ( 'NONE',  ( -4.350000000000023626, 2.500000000000000000, 6.841600689897072485 ) ) ;
#129219=EDGE_LOOP ( 'NONE', ( #16767, #59514 ) ) ;
#129220=CARTESIAN_POINT ( 'NONE',  ( 18.46077503349216187, -0.2574728941692127626, 4.048716373199397367 ) ) ;
#129221=ADVANCED_FACE ( 'NONE', ( #19010 ), #108200, .T. ) ;
#129222=ORIENTED_EDGE ( 'NONE', *, *, #83512, .F. ) ;
#129223=CARTESIAN_POINT ( 'NONE',  ( 9.999999999999952038, 2.500000000000000000, -0.1000000000000022815 ) ) ;
#129224=DIRECTION ( 'NONE',  ( 0.000000000000000000, 1.000000000000000000, 0.000000000000000000 ) ) ;
#129225=ORIENTED_EDGE ( 'NONE', *, *, #74349, .T. ) ;
#129226=DIRECTION ( 'NONE',  ( -0.000000000000000000, 1.000000000000000000, -0.000000000000000000 ) ) ;
#129227=AXIS2_PLACEMENT_3D ( 'NONE', #29339, #39811, #77760 ) ;
#129228=DIRECTION ( 'NONE',  ( -0.000000000000000000, 1.000000000000000000, -0.000000000000000000 ) ) ;
#129229=ORIENTED_EDGE ( 'NONE', *, *, #53015, .T. ) ;
#129230=AXIS2_PLACEMENT_3D ( 'NONE', #19039, #77975, #77333 ) ;
#129231=CARTESIAN_POINT ( 'NONE',  ( -8.749999999999975131, 2.500000000000000000, -2.165063509461101710 ) ) ;
#129232=EDGE_LOOP ( 'NONE', ( #54131, #43768, #4057, #32733 ) ) ;
#129233=ADVANCED_FACE ( 'NONE', ( #114331 ), #73127, .T. ) ;
#129234=ADVANCED_FACE ( 'NONE', ( #84218 ), #24672, .T. ) ;
#129235=ORIENTED_EDGE ( 'NONE', *, *, #95818, .T. ) ;
#129236=CARTESIAN_POINT ( 'NONE',  ( -4.600000000000028066, 12.50000000000000000, -3.637306695894650055 ) ) ;
#129237=CARTESIAN_POINT ( 'NONE',  ( -2.900000000000029221, 12.50000000000000000, -5.088040615133791356 ) ) ;
#129238=EDGE_CURVE ( 'NONE', #61247, #91045, #82954, .T. ) ;
#129239=CARTESIAN_POINT ( 'NONE',  ( 10.19999999999991225, 2.500000000000000000, 3.883716857408420431 ) ) ;
#129241=CARTESIAN_POINT ( 'NONE',  ( -12.09999999999999609, 2.500000000000000000, 0.5928203230275536084 ) ) ;
#129242=CARTESIAN_POINT ( 'NONE',  ( 3.349999999999945466, 2.500000000000000000, -6.395190528383301931 ) ) ;
#129243=CIRCLE ( 'NONE', #79054, 0.06509327318403745899 ) ;
#129244=VERTEX_POINT ( 'NONE', #27888 ) ;
#129245=CARTESIAN_POINT ( 'NONE',  ( 2.899999999999946620, 12.50000000000000000, 0.6928203230275494784 ) ) ;
#129246=EDGE_CURVE ( 'NONE', #94085, #122392, #37119, .T. ) ;
#129247=ORIENTED_EDGE ( 'NONE', *, *, #72595, .T. ) ;
#129248=ADVANCED_FACE ( 'NONE', ( #8239 ), #11469, .T. ) ;
#129249=DIRECTION ( 'NONE',  ( 0.000000000000000000, -0.9999939076577903929, 0.003490651415223739937 ) ) ;
#129250=CARTESIAN_POINT ( 'NONE',  ( -3.100000000000028511, 2.500000000000000000, -4.576537180435977348 ) ) ;
#129251=AXIS2_PLACEMENT_3D ( 'NONE', #66025, #55570, #98062 ) ;
#129252=EDGE_CURVE ( 'NONE', #75374, #24991, #97740, .T. ) ;
#129253=VECTOR ( 'NONE', #68183, 1000.000000000000000 ) ;
#129255=DIRECTION ( 'NONE',  ( 0.000000000000000000, 0.000000000000000000, -1.000000000000000000 ) ) ;
#129256=DIRECTION ( 'NONE',  ( -0.000000000000000000, -1.000000000000000000, -0.000000000000000000 ) ) ;
#129257=DIRECTION ( 'NONE',  ( 0.000000000000000000, 0.000000000000000000, 1.000000000000000000 ) ) ;
#129258=DIRECTION ( 'NONE',  ( 0.000000000000000000, 0.000000000000000000, 1.000000000000000000 ) ) ;
#129259=VERTEX_POINT ( 'NONE', #51422 ) ;
#129260=CIRCLE ( 'NONE', #110439, 0.06509327318403745899 ) ;
#129261=PLANE ( 'NONE',  #94050 ) ;
#129262=DIRECTION ( 'NONE',  ( 0.000000000000000000, 0.000000000000000000, 1.000000000000000000 ) ) ;
#129264=CIRCLE ( 'NONE', #108297, 0.06509327318403745899 ) ;
#129265=ORIENTED_EDGE ( 'NONE', *, *, #54070, .F. ) ;
#129266=AXIS2_PLACEMENT_3D ( 'NONE', #91339, #89412, #29849 ) ;
#129267=FACE_OUTER_BOUND ( 'NONE', #106618, .T. ) ;
#129268=CONICAL_SURFACE ( 'NONE', #72815, 0.1000000000000002554, 0.003490658503988666988 ) ;
#129269=ORIENTED_EDGE ( 'NONE', *, *, #26374, .T. ) ;
#129270=VERTEX_POINT ( 'NONE', #101797 ) ;
#129271=CARTESIAN_POINT ( 'NONE',  ( 4.599999999999937472, 12.50000000000000000, 0.6928203230275494784 ) ) ;
#129272=ORIENTED_EDGE ( 'NONE', *, *, #87837, .F. ) ;
#129273=CARTESIAN_POINT ( 'NONE',  ( -7.300000000000016698, 12.50000000000000000, -4.741630453620016006 ) ) ;
#129274=CARTESIAN_POINT ( 'NONE',  ( -4.350000000000027178, 2.500000000000000000, -6.048780366869526581 ) ) ;
#129275=ORIENTED_EDGE ( 'NONE', *, *, #110709, .T. ) ;
#129276=CARTESIAN_POINT ( 'NONE',  ( -7.700000000000016165, 12.50000000000000000, 0.2813168883297361700 ) ) ;
#129277=DIRECTION ( 'NONE',  ( -0.000000000000000000, -1.000000000000000000, -0.000000000000000000 ) ) ;
#129278=ORIENTED_EDGE ( 'NONE', *, *, #103796, .T. ) ;
#129279=DIRECTION ( 'NONE',  ( 0.000000000000000000, 0.000000000000000000, 1.000000000000000000 ) ) ;
#129280=AXIS2_PLACEMENT_3D ( 'NONE', #11599, #89515, #9668 ) ;
#129281=DIRECTION ( 'NONE',  ( -0.000000000000000000, 1.000000000000000000, -0.000000000000000000 ) ) ;
#129282=EDGE_LOOP ( 'NONE', ( #20683, #68483 ) ) ;
#129283=EDGE_CURVE ( 'NONE', #36770, #84687, #85224, .T. ) ;
#129284=CONICAL_SURFACE ( 'NONE', #64412, 0.1000000000000000472, 0.003490658503988666988 ) ;
#129285=AXIS2_PLACEMENT_3D ( 'NONE', #70168, #9954, #70800 ) ;
#129286=VERTEX_POINT ( 'NONE', #42235 ) ;
#129287=EDGE_CURVE ( 'NONE', #4055, #51156, #89428, .T. ) ;
#129288=VERTEX_POINT ( 'NONE', #112900 ) ;
#129289=DIRECTION ( 'NONE',  ( -0.000000000000000000, 1.000000000000000000, -0.000000000000000000 ) ) ;
#129290=DIRECTION ( 'NONE',  ( 0.000000000000000000, 0.000000000000000000, -1.000000000000000000 ) ) ;
#129291=DIRECTION ( 'NONE',  ( -0.000000000000000000, -1.000000000000000000, -0.000000000000000000 ) ) ;
#129292=FACE_BOUND ( 'NONE', #21275, .T. ) ;
#129293=ORIENTED_EDGE ( 'NONE', *, *, #58006, .F. ) ;
#129294=DIRECTION ( 'NONE',  ( 0.000000000000000000, 0.000000000000000000, 1.000000000000000000 ) ) ;
#129295=DIRECTION ( 'NONE',  ( 0.000000000000000000, 0.000000000000000000, -1.000000000000000000 ) ) ;
#129296=ORIENTED_EDGE ( 'NONE', *, *, #121965, .T. ) ;
#129297=ADVANCED_FACE ( 'NONE', ( #12739 ), #82809, .T. ) ;
#129298=CARTESIAN_POINT ( 'NONE',  ( -4.600000000000028955, 12.50000000000000000, -4.395220292106239768 ) ) ;
#129299=DIRECTION ( 'NONE',  ( 0.000000000000000000, -0.000000000000000000, 1.000000000000000000 ) ) ;
#129300=LINE ( 'NONE', #21242, #42337 ) ;
#129301=DIRECTION ( 'NONE',  ( 0.000000000000000000, 0.000000000000000000, -1.000000000000000000 ) ) ;
#129302=CARTESIAN_POINT ( 'NONE',  ( -4.400000000000028777, 2.500000000000000000, -4.676537180435978769 ) ) ;
#129303=DIRECTION ( 'NONE',  ( -4.274815082592931898E-19, -0.9999939076577903929, -0.003490651415223739937 ) ) ;
#129304=CARTESIAN_POINT ( 'NONE',  ( 0.8499999999999553468, 2.500000000000000000, -2.265063509461101798 ) ) ;
#129305=CONICAL_SURFACE ( 'NONE', #51930, 0.09999999999999982514, 0.003490658503988666988 ) ;
#129306=CIRCLE ( 'NONE', #8275, 0.09999999999999999167 ) ;
#129307=ORIENTED_EDGE ( 'NONE', *, *, #58044, .T. ) ;
#129308=ORIENTED_EDGE ( 'NONE', *, *, #91409, .T. ) ;
#129309=EDGE_LOOP ( 'NONE', ( #76691, #44499, #110491, #119022 ) ) ;
#129310=AXIS2_PLACEMENT_3D ( 'NONE', #71875, #92134, #42414 ) ;
#129311=ORIENTED_EDGE ( 'NONE', *, *, #66525, .T. ) ;
#129312=VERTEX_POINT ( 'NONE', #31137 ) ;
#129313=DIRECTION ( 'NONE',  ( 0.000000000000000000, -0.000000000000000000, 1.000000000000000000 ) ) ;
#129314=DIRECTION ( 'NONE',  ( 0.000000000000000000, -0.000000000000000000, 1.000000000000000000 ) ) ;
#129315=ORIENTED_EDGE ( 'NONE', *, *, #27662, .T. ) ;
#129316=FACE_BOUND ( 'NONE', #101264, .T. ) ;
#129317=CARTESIAN_POINT ( 'NONE',  ( -12.09999999999999432, 12.50000000000000000, 3.637306695894644726 ) ) ;
#129318=AXIS2_PLACEMENT_3D ( 'NONE', #95678, #57018, #97599 ) ;
#129319=VECTOR ( 'NONE', #15660, 1000.000000000000000 ) ;
#129320=AXIS2_PLACEMENT_3D ( 'NONE', #61633, #11862, #41988 ) ;
#129321=DIRECTION ( 'NONE',  ( 0.000000000000000000, 1.000000000000000000, 0.000000000000000000 ) ) ;
#129322=CARTESIAN_POINT ( 'NONE',  ( 12.89999999999989910, 2.500000000000000000, 0.6928203230275494784 ) ) ;
#129323=PLANE ( 'NONE',  #45457 ) ;
#129324=DIRECTION ( 'NONE',  ( -0.000000000000000000, 1.000000000000000000, -0.000000000000000000 ) ) ;
#129325=CARTESIAN_POINT ( 'NONE',  ( 3.349999999999942801, 12.50000000000000000, 2.792790559304612064 ) ) ;
#129326=ORIENTED_EDGE ( 'NONE', *, *, #54680, .T. ) ;
#129327=AXIS2_PLACEMENT_3D ( 'NONE', #27327, #17514, #10897 ) ;
#129328=ORIENTED_EDGE ( 'NONE', *, *, #94049, .T. ) ;
#129329=AXIS2_PLACEMENT_3D ( 'NONE', #56902, #64805, #104718 ) ;
#129330=EDGE_CURVE ( 'NONE', #86526, #74427, #62253, .T. ) ;
#129331=ORIENTED_EDGE ( 'NONE', *, *, #89783, .T. ) ;
#129332=VERTEX_POINT ( 'NONE', #63149 ) ;
#129333=CARTESIAN_POINT ( 'NONE',  ( 10.63722763359408319, 2.500000000000000444, 8.014330155125131583 ) ) ;
#129334=DIRECTION ( 'NONE',  ( 0.000000000000000000, 0.000000000000000000, 1.000000000000000000 ) ) ;
#129335=EDGE_LOOP ( 'NONE', ( #91163, #73307 ) ) ;
#129336=LINE ( 'NONE', #119474, #62281 ) ;
#129337=CONICAL_SURFACE ( 'NONE', #54092, 0.1000000000000002554, 0.003490658503988666988 ) ;
#129338=CARTESIAN_POINT ( 'NONE',  ( -1.250000000000037970, 2.500000000000000000, 2.857883832488649301 ) ) ;
#129339=DIRECTION ( 'NONE',  ( 0.000000000000000000, 0.000000000000000000, 1.000000000000000000 ) ) ;
#129340=CIRCLE ( 'NONE', #85400, 0.06509327318403741736 ) ;
#129341=CARTESIAN_POINT ( 'NONE',  ( 5.599999999999933031, 2.500000000000000000, -0.3464101615137783474 ) ) ;
#129342=CARTESIAN_POINT ( 'NONE',  ( 6.649999999999931966, 2.500000000000000000, -5.902370205355750521 ) ) ;
#129343=DIRECTION ( 'NONE',  ( -4.274815082592931898E-19, -0.9999939076577903929, -0.003490651415223739937 ) ) ;
#129344=EDGE_CURVE ( 'NONE', #59339, #80261, #82152, .T. ) ;
#129345=AXIS2_PLACEMENT_3D ( 'NONE', #56737, #96671, #7652 ) ;
#129347=ADVANCED_FACE ( 'NONE', ( #52687 ), #54606, .T. ) ;
#129348=VERTEX_POINT ( 'NONE', #114189 ) ;
#129349=CARTESIAN_POINT ( 'NONE',  ( 3.949999999999942446, 2.500000000000000000, -6.741600689897078169 ) ) ;
#129350=CONICAL_SURFACE ( 'NONE', #112606, 0.1000000000000002554, 0.003490658503988666988 ) ;
#129351=ORIENTED_EDGE ( 'NONE', *, *, #59304, .T. ) ;
#129352=VERTEX_POINT ( 'NONE', #85366 ) ;
#129354=CARTESIAN_POINT ( 'NONE',  ( -8.750000000000008882, 2.500000000000000000, -2.857883832488653741 ) ) ;
#129355=CARTESIAN_POINT ( 'NONE',  ( 3.299999999999944755, 2.500000000000000000, -2.385244779468109755E-15 ) ) ;
#129356=CARTESIAN_POINT ( 'NONE',  ( -3.749999999999994671, 12.50000000000000000, -6.495190528383302464 ) ) ;
#129357=EDGE_CURVE ( 'NONE', #127183, #114003, #84720, .T. ) ;
#129358=ORIENTED_EDGE ( 'NONE', *, *, #57135, .F. ) ;
#129359=AXIS2_PLACEMENT_3D ( 'NONE', #44170, #42918, #124676 ) ;
#129360=VERTEX_POINT ( 'NONE', #124659 ) ;
#129361=DIRECTION ( 'NONE',  ( -0.000000000000000000, 1.000000000000000000, -0.000000000000000000 ) ) ;
#129362=CONICAL_SURFACE ( 'NONE', #45721, 0.1000000000000002554, 0.003490658503988666988 ) ;
#129363=CARTESIAN_POINT ( 'NONE',  ( -3.950000000000024603, 12.50000000000000000, 1.818653347947321475 ) ) ;
#129364=CARTESIAN_POINT ( 'NONE',  ( 0.5999999999999560130, 2.500000000000000000, -4.083716857408426826 ) ) ;
#129365=CARTESIAN_POINT ( 'NONE',  ( -11.89999999999999680, 12.50000000000000000, -0.3464101615137741841 ) ) ;
#129366=ORIENTED_EDGE ( 'NONE', *, *, #58252, .F. ) ;
#129368=AXIS2_PLACEMENT_3D ( 'NONE', #3405, #62341, #13859 ) ;
#129369=ORIENTED_EDGE ( 'NONE', *, *, #911, .T. ) ;
#129370=CARTESIAN_POINT ( 'NONE',  ( -5.650000000000019895, 2.500000000000000000, 1.718653347947321386 ) ) ;
#129371=ORIENTED_EDGE ( 'NONE', *, *, #25247, .T. ) ;
#129372=CARTESIAN_POINT ( 'NONE',  ( 3.149999999999944400, 2.500000000000000000, 1.718653347947321386 ) ) ;
#129373=ADVANCED_FACE ( 'NONE', ( #35006 ), #55967, .T. ) ;
#129374=CIRCLE ( 'NONE', #108495, 0.1000000000000000056 ) ;
#129375=CIRCLE ( 'NONE', #64584, 0.06509327318403741736 ) ;
#129376=DIRECTION ( 'NONE',  ( 0.000000000000000000, 0.000000000000000000, 1.000000000000000000 ) ) ;
#129377=FACE_OUTER_BOUND ( 'NONE', #98995, .T. ) ;
#129378=CONICAL_SURFACE ( 'NONE', #3948, 0.09999999999999982514, 0.003490658503988666988 ) ;
#129379=CARTESIAN_POINT ( 'NONE',  ( -1.900000000000034550, 2.500000000000000000, 4.776537180435972196 ) ) ;
#129380=ORIENTED_EDGE ( 'NONE', *, *, #53007, .T. ) ;
#129381=ADVANCED_FACE ( 'NONE', ( #74265 ), #53832, .T. ) ;
#129382=DIRECTION ( 'NONE',  ( 0.000000000000000000, 1.000000000000000000, 0.000000000000000000 ) ) ;
#129383=CONICAL_SURFACE ( 'NONE', #72915, 0.09999999999999982514, 0.003490658503988666988 ) ;
#129384=CIRCLE ( 'NONE', #89646, 0.06509327318403745899 ) ;
#129385=VERTEX_POINT ( 'NONE', #74909 ) ;
#129386=ORIENTED_EDGE ( 'NONE', *, *, #111349, .T. ) ;
#129387=ADVANCED_FACE ( 'NONE', ( #84070 ), #39290, .T. ) ;
#129388=ADVANCED_FACE ( 'NONE', ( #114815 ), #129171, .T. ) ;
#129389=DIRECTION ( 'NONE',  ( -0.000000000000000000, 1.000000000000000000, -0.000000000000000000 ) ) ;
#129390=DIRECTION ( 'NONE',  ( 0.000000000000000000, 1.000000000000000000, 0.000000000000000000 ) ) ;
#129391=DIRECTION ( 'NONE',  ( 0.000000000000000000, 1.000000000000000000, 0.000000000000000000 ) ) ;
#129392=EDGE_CURVE ( 'NONE', #118832, #45708, #55272, .T. ) ;
#129394=ADVANCED_FACE ( 'NONE', ( #65722 ), #99804, .T. ) ;
#129395=DIRECTION ( 'NONE',  ( 0.000000000000000000, 0.000000000000000000, 1.000000000000000000 ) ) ;
#129396=CARTESIAN_POINT ( 'NONE',  ( -6.249999999999984901, 12.50000000000000000, -2.165063509461101710 ) ) ;
#129397=PLANE ( 'NONE',  #19725 ) ;
#129398=CARTESIAN_POINT ( 'NONE',  ( -2.300000000000032685, 2.500000000000000000, -0.4464101615137783252 ) ) ;
#129399=CARTESIAN_POINT ( 'NONE',  ( 9.199999999999915801, 12.50000000000000000, 4.330127018922196314 ) ) ;
#129400=EDGE_CURVE ( 'NONE', #47255, #62375, #85988, .T. ) ;
#129401=VECTOR ( 'NONE', #117661, 1000.000000000000000 ) ;
#129402=EDGE_CURVE ( 'NONE', #61169, #53570, #81025, .T. ) ;
#129403=EDGE_CURVE ( 'NONE', #92009, #35838, #59146, .T. ) ;
#129404=ADVANCED_FACE ( 'NONE', ( #29673 ), #74768, .T. ) ;
#129405=AXIS2_PLACEMENT_3D ( 'NONE', #78830, #40842, #33428 ) ;
#129406=EDGE_LOOP ( 'NONE', ( #68758, #34405 ) ) ;
#129407=CARTESIAN_POINT ( 'NONE',  ( 6.049999999999932321, 12.50000000000000000, -1.883746621131363597 ) ) ;
#129408=CARTESIAN_POINT ( 'NONE',  ( 15.19999999999989093, 2.500000000000000000, 0.4464101615137735513 ) ) ;
#129409=CARTESIAN_POINT ( 'NONE',  ( 1.849999999999949685, 12.50000000000000000, -2.511473670974877948 ) ) ;
#129410=CARTESIAN_POINT ( 'NONE',  ( 9.399999999999918643, 12.50000000000000000, -0.3464101615137782364 ) ) ;
#129411=DIRECTION ( 'NONE',  ( -0.000000000000000000, -1.000000000000000000, -0.000000000000000000 ) ) ;
#129412=ADVANCED_FACE ( 'NONE', ( #17907 ), #127098, .T. ) ;
#129413=AXIS2_PLACEMENT_3D ( 'NONE', #68351, #70936, #60494 ) ;
#129414=ORIENTED_EDGE ( 'NONE', *, *, #25571, .F. ) ;
#129415=VECTOR ( 'NONE', #39224, 1000.000000000000000 ) ;
#129416=LINE ( 'NONE', #409, #86332 ) ;
#129417=AXIS2_PLACEMENT_3D ( 'NONE', #54162, #15504, #55445 ) ;
#129418=DIRECTION ( 'NONE',  ( 0.000000000000000000, 0.000000000000000000, 1.000000000000000000 ) ) ;
#129419=DIRECTION ( 'NONE',  ( 0.000000000000000000, -0.000000000000000000, 1.000000000000000000 ) ) ;
#129420=VERTEX_POINT ( 'NONE', #99713 ) ;
#129421=CONICAL_SURFACE ( 'NONE', #52039, 0.1000000000000000472, 0.003490658503988666988 ) ;
#129422=ORIENTED_EDGE ( 'NONE', *, *, #14070, .F. ) ;
#129423=CARTESIAN_POINT ( 'NONE',  ( 3.099999999999945022, 12.50000000000000000, -4.676537180435978769 ) ) ;
#129424=VECTOR ( 'NONE', #94119, 1000.000000000000000 ) ;
#129425=ORIENTED_EDGE ( 'NONE', *, *, #39476, .F. ) ;
#129426=EDGE_LOOP ( 'NONE', ( #1322, #73390, #28052, #94179 ) ) ;
#129427=EDGE_LOOP ( 'NONE', ( #40312, #127132 ) ) ;
#129428=FACE_OUTER_BOUND ( 'NONE', #125582, .T. ) ;
#129429=CARTESIAN_POINT ( 'NONE',  ( 6.649999999999928413, 2.500000000000000000, 2.857883832488649301 ) ) ;
#129430=DIRECTION ( 'NONE',  ( 0.000000000000000000, 1.000000000000000000, 0.000000000000000000 ) ) ;
#129431=DIRECTION ( 'NONE',  ( -0.000000000000000000, 1.000000000000000000, -0.000000000000000000 ) ) ;
#129432=AXIS2_PLACEMENT_3D ( 'NONE', #120622, #9148, #98810 ) ;
#129433=ORIENTED_EDGE ( 'NONE', *, *, #95685, .F. ) ;
#129434=FACE_OUTER_BOUND ( 'NONE', #99920, .T. ) ;
#129435=EDGE_LOOP ( 'NONE', ( #129010, #12628 ) ) ;
#129436=CIRCLE ( 'NONE', #22900, 0.06509327318403741736 ) ;
#129437=DIRECTION ( 'NONE',  ( 0.000000000000000000, -0.000000000000000000, 1.000000000000000000 ) ) ;
#129438=CARTESIAN_POINT ( 'NONE',  ( 14.34999999999989306, 2.500000000000000000, -2.511473670974877948 ) ) ;
#129439=DIRECTION ( 'NONE',  ( 0.000000000000000000, 1.000000000000000000, 0.000000000000000000 ) ) ;
#129440=LINE ( 'NONE', #40402, #12063 ) ;
#129441=EDGE_LOOP ( 'NONE', ( #10723, #50857 ) ) ;
#129442=EDGE_CURVE ( 'NONE', #123754, #16842, #3743, .T. ) ;
#129443=AXIS2_PLACEMENT_3D ( 'NONE', #18104, #27931, #50170 ) ;
#129444=ORIENTED_EDGE ( 'NONE', *, *, #51468, .T. ) ;
#129445=ORIENTED_EDGE ( 'NONE', *, *, #83225, .T. ) ;
#129446=EDGE_LOOP ( 'NONE', ( #101991, #67164 ) ) ;
#129447=ADVANCED_FACE ( 'NONE', ( #8715 ), #57856, .T. ) ;
#129448=ORIENTED_EDGE ( 'NONE', *, *, #80019, .F. ) ;
#129449=DIRECTION ( 'NONE',  ( 0.000000000000000000, 0.000000000000000000, 1.000000000000000000 ) ) ;
#129450=DIRECTION ( 'NONE',  ( 0.000000000000000000, 0.000000000000000000, -1.000000000000000000 ) ) ;
#129451=DIRECTION ( 'NONE',  ( -0.000000000000000000, 1.000000000000000000, -0.000000000000000000 ) ) ;
#129452=FACE_BOUND ( 'NONE', #111433, .T. ) ;
#129453=CARTESIAN_POINT ( 'NONE',  ( -2.100000000000033396, 2.500000000000000000, -0.5928203230275542746 ) ) ;
#129454=FACE_OUTER_BOUND ( 'NONE', #20043, .T. ) ;
#129455=CIRCLE ( 'NONE', #29186, 0.1000000000000000472 ) ;
#129456=DIRECTION ( 'NONE',  ( 0.000000000000000000, 1.000000000000000000, 0.000000000000000000 ) ) ;
#129457=DIRECTION ( 'NONE',  ( -0.000000000000000000, -1.000000000000000000, -0.000000000000000000 ) ) ;
#129458=AXIS2_PLACEMENT_3D ( 'NONE', #36379, #35716, #124738 ) ;
#129459=CARTESIAN_POINT ( 'NONE',  ( 105.5000000000000142, 2.449293598294706414E-16, -2.000000000000000000 ) ) ;
#129460=DIRECTION ( 'NONE',  ( 0.000000000000000000, 1.000000000000000000, 0.000000000000000000 ) ) ;
#129461=VECTOR ( 'NONE', #71043, 1000.000000000000000 ) ;
#129462=CARTESIAN_POINT ( 'NONE',  ( 7.499999999999927169, 12.50000000000000000, -4.957854068765716882 ) ) ;
#129463=DIRECTION ( 'NONE',  ( 0.000000000000000000, 0.000000000000000000, 1.000000000000000000 ) ) ;
#129464=AXIS2_PLACEMENT_3D ( 'NONE', #41667, #61938, #101853 ) ;
#129465=AXIS2_PLACEMENT_3D ( 'NONE', #89656, #21558, #81753 ) ;
#129466=EDGE_LOOP ( 'NONE', ( #27494, #5909 ) ) ;
#129467=ORIENTED_EDGE ( 'NONE', *, *, #5337, .T. ) ;
#129468=ORIENTED_EDGE ( 'NONE', *, *, #29029, .T. ) ;
#129469=ORIENTED_EDGE ( 'NONE', *, *, #58127, .F. ) ;
#129470=DIRECTION ( 'NONE',  ( 0.000000000000000000, 1.000000000000000000, 0.000000000000000000 ) ) ;
#129471=AXIS2_PLACEMENT_3D ( 'NONE', #61852, #90650, #59931 ) ;
#129472=CARTESIAN_POINT ( 'NONE',  ( 14.14999999999989733, 2.500000000000000000, 2.757883832488649656 ) ) ;
#129473=FACE_BOUND ( 'NONE', #16841, .T. ) ;
#129474=PLANE ( 'NONE',  #49951 ) ;
#129475=CONICAL_SURFACE ( 'NONE', #73011, 0.1000000000000002554, 0.003490658503988666988 ) ;
#129476=CIRCLE ( 'NONE', #54138, 0.09999999999999982514 ) ;
#129477=VERTEX_POINT ( 'NONE', #40142 ) ;
#129478=DIRECTION ( 'NONE',  ( 0.000000000000000000, 0.000000000000000000, 1.000000000000000000 ) ) ;
#129479=CARTESIAN_POINT ( 'NONE',  ( -3.550000000000031797, 12.50000000000000000, -6.148780366869526226 ) ) ;
#129480=LINE ( 'NONE', #1140, #15532 ) ;
#129481=CARTESIAN_POINT ( 'NONE',  ( 11.24999999999994493, 2.500000000000000000, 6.595190528383296780 ) ) ;
#129482=ORIENTED_EDGE ( 'NONE', *, *, #56071, .T. ) ;
#129484=ADVANCED_FACE ( 'NONE', ( #8087 ), #51880, .T. ) ;
#129485=EDGE_LOOP ( 'NONE', ( #23737, #54616, #42714, #73466 ) ) ;
#129486=VERTEX_POINT ( 'NONE', #98395 ) ;
#129487=AXIS2_PLACEMENT_3D ( 'NONE', #24491, #96433, #84039 ) ;
#129488=DIRECTION ( 'NONE',  ( -4.274815082592931898E-19, -0.9999939076577903929, -0.003490651415223739937 ) ) ;
#129489=DIRECTION ( 'NONE',  ( -0.000000000000000000, -1.000000000000000000, -0.000000000000000000 ) ) ;
#129490=ORIENTED_EDGE ( 'NONE', *, *, #105107, .F. ) ;
#129491=CIRCLE ( 'NONE', #50068, 0.06509327318403745899 ) ;
#129492=CARTESIAN_POINT ( 'NONE',  ( -6.250000000000015987, 2.500000000000000000, 5.702370205355745014 ) ) ;
#129493=AXIS2_PLACEMENT_3D ( 'NONE', #34061, #5227, #45177 ) ;
#129494=CARTESIAN_POINT ( 'NONE',  ( 1.649999999999951950, 2.500000000000000000, -5.902370205355750521 ) ) ;
#129495=EDGE_LOOP ( 'NONE', ( #96275, #2717, #55887, #118037 ) ) ;
#129496=CARTESIAN_POINT ( 'NONE',  ( 7.899999999999924860, 2.500000000000000000, -3.637306695894650055 ) ) ;
#129497=ORIENTED_EDGE ( 'NONE', *, *, #112519, .F. ) ;
#129498=EDGE_CURVE ( 'NONE', #109985, #84685, #119332, .T. ) ;
#129499=EDGE_CURVE ( 'NONE', #88412, #61414, #93637, .T. ) ;
#129500=CARTESIAN_POINT ( 'NONE',  ( -12.09999999999999609, 2.500000000000000000, 4.330127018922196314 ) ) ;
#129501=EDGE_LOOP ( 'NONE', ( #122885, #61958 ) ) ;
#129502=DIRECTION ( 'NONE',  ( 0.000000000000000000, 0.000000000000000000, 1.000000000000000000 ) ) ;
#129503=FACE_BOUND ( 'NONE', #42834, .T. ) ;
#129504=CIRCLE ( 'NONE', #121063, 0.1000000000000002554 ) ;
#129505=ORIENTED_EDGE ( 'NONE', *, *, #64542, .F. ) ;
#129507=ORIENTED_EDGE ( 'NONE', *, *, #13405, .T. ) ;
#129508=DIRECTION ( 'NONE',  ( -0.000000000000000000, -1.000000000000000000, -0.000000000000000000 ) ) ;
#129509=DIRECTION ( 'NONE',  ( -0.000000000000000000, -1.000000000000000000, -0.000000000000000000 ) ) ;
#129510=DIRECTION ( 'NONE',  ( 0.000000000000000000, 0.000000000000000000, 1.000000000000000000 ) ) ;
#129512=ADVANCED_FACE ( 'NONE', ( #109528 ), #67651, .T. ) ;
#129513=CARTESIAN_POINT ( 'NONE',  ( -10.00000000000000355, 12.50000000000000000, 3.572213422710607489 ) ) ;
#129514=AXIS2_PLACEMENT_3D ( 'NONE', #112849, #34944, #4801 ) ;
#129515=VERTEX_POINT ( 'NONE', #87922 ) ;
#129516=ORIENTED_EDGE ( 'NONE', *, *, #93320, .F. ) ;
#129517=AXIS2_PLACEMENT_3D ( 'NONE', #3492, #22510, #53883 ) ;
#129518=ORIENTED_EDGE ( 'NONE', *, *, #56074, .F. ) ;
#129519=DIRECTION ( 'NONE',  ( 0.000000000000000000, -0.000000000000000000, 1.000000000000000000 ) ) ;
#129521=DIRECTION ( 'NONE',  ( 0.000000000000000000, 0.000000000000000000, 1.000000000000000000 ) ) ;
#129522=VERTEX_POINT ( 'NONE', #19861 ) ;
#129523=ORIENTED_EDGE ( 'NONE', *, *, #17031, .F. ) ;
#129525=CARTESIAN_POINT ( 'NONE',  ( -10.85000000000000142, 12.50000000000000000, -2.922977105672687426 ) ) ;
#129526=VERTEX_POINT ( 'NONE', #97765 ) ;
#129527=FACE_OUTER_BOUND ( 'NONE', #71863, .T. ) ;
#129529=PLANE ( 'NONE',  #28131 ) ;
#129530=DIRECTION ( 'NONE',  ( -4.274815082592931898E-19, -0.9999939076577903929, -0.003490651415223739937 ) ) ;
#129531=DIRECTION ( 'NONE',  ( -0.000000000000000000, -1.000000000000000000, -0.000000000000000000 ) ) ;
#129533=AXIS2_PLACEMENT_3D ( 'NONE', #93114, #103576, #71518 ) ;
#129534=CARTESIAN_POINT ( 'NONE',  ( -4.150000000000027889, 2.500000000000000000, -7.088010851410853519 ) ) ;
#129535=DIRECTION ( 'NONE',  ( 0.000000000000000000, 1.000000000000000000, 0.000000000000000000 ) ) ;
#129536=VERTEX_POINT ( 'NONE', #48675 ) ;
#129537=VERTEX_POINT ( 'NONE', #78140 ) ;
#129538=EDGE_CURVE ( 'NONE', #95183, #43428, #76908, .T. ) ;
#129539=DIRECTION ( 'NONE',  ( -0.000000000000000000, -1.000000000000000000, -0.000000000000000000 ) ) ;
#129540=ORIENTED_EDGE ( 'NONE', *, *, #61817, .F. ) ;
#129541=VERTEX_POINT ( 'NONE', #68296 ) ;
#129542=EDGE_CURVE ( 'NONE', #120092, #92046, #48036, .T. ) ;
#129544=CARTESIAN_POINT ( 'NONE',  ( 9.149999999999915090, 12.50000000000000000, -2.230156782645139391 ) ) ;
#129545=CARTESIAN_POINT ( 'NONE',  ( -11.64999999999999680, 12.50000000000000000, -7.188010851410850499 ) ) ;
#129546=ADVANCED_FACE ( 'NONE', ( #70246 ), #102046, .T. ) ;
#129547=DIRECTION ( 'NONE',  ( -0.000000000000000000, 1.000000000000000000, -0.000000000000000000 ) ) ;
#129548=DIRECTION ( 'NONE',  ( 0.000000000000000000, 0.000000000000000000, 1.000000000000000000 ) ) ;
#129549=DIRECTION ( 'NONE',  ( -0.000000000000000000, 1.000000000000000000, -0.000000000000000000 ) ) ;
#129550=PLANE ( 'NONE',  #87448 ) ;
#129552=ADVANCED_FACE ( 'NONE', ( #128548 ), #78794, .T. ) ;
#129553=AXIS2_PLACEMENT_3D ( 'NONE', #31614, #40808, #51903 ) ;
#129554=EDGE_CURVE ( 'NONE', #113501, #94166, #62999, .T. ) ;
#129555=DIRECTION ( 'NONE',  ( -0.000000000000000000, 1.000000000000000000, -0.000000000000000000 ) ) ;
#129556=ORIENTED_EDGE ( 'NONE', *, *, #119415, .T. ) ;
#129557=AXIS2_PLACEMENT_3D ( 'NONE', #57423, #18773, #97338 ) ;
#129558=AXIS2_PLACEMENT_3D ( 'NONE', #126854, #37192, #98024 ) ;
#129559=EDGE_CURVE ( 'NONE', #90845, #48001, #45623, .T. ) ;
#129560=ORIENTED_EDGE ( 'NONE', *, *, #112312, .T. ) ;
#129561=AXIS2_PLACEMENT_3D ( 'NONE', #74884, #44129, #63782 ) ;
#129562=ORIENTED_EDGE ( 'NONE', *, *, #41038, .F. ) ;
#129563=ORIENTED_EDGE ( 'NONE', *, *, #103474, .T. ) ;
#129564=CARTESIAN_POINT ( 'NONE',  ( -5.450000000000019718, 2.500000000000000000, 2.165063509461097713 ) ) ;
#129565=CARTESIAN_POINT ( 'NONE',  ( -11.84999999999999609, 2.500000000000000000, 2.411473670974873862 ) ) ;
#129566=EDGE_CURVE ( 'NONE', #74274, #91624, #41427, .T. ) ;
#129567=CIRCLE ( 'NONE', #1988, 0.1000000000000002554 ) ;
#129568=AXIS2_PLACEMENT_3D ( 'NONE', #35713, #67741, #107676 ) ;
#129569=EDGE_LOOP ( 'NONE', ( #31833, #88252 ) ) ;
#129570=DIRECTION ( 'NONE',  ( 0.000000000000000000, -0.000000000000000000, 1.000000000000000000 ) ) ;
#129571=DIRECTION ( 'NONE',  ( 0.000000000000000000, 0.000000000000000000, 1.000000000000000000 ) ) ;
#129572=LINE ( 'NONE', #20235, #32651 ) ;
#129573=CARTESIAN_POINT ( 'NONE',  ( 11.04999999999991012, 12.50000000000000000, 6.776507416713035248 ) ) ;
#129574=EDGE_LOOP ( 'NONE', ( #129497, #67311, #60689, #108216 ) ) ;
#129575=DIRECTION ( 'NONE',  ( -0.000000000000000000, 1.000000000000000000, -0.000000000000000000 ) ) ;
#129576=CARTESIAN_POINT ( 'NONE',  ( 4.599999999999936584, 2.500000000000000000, 4.430127018922196847 ) ) ;
#129577=VERTEX_POINT ( 'NONE', #856 ) ;
#129578=ORIENTED_EDGE ( 'NONE', *, *, #93946, .F. ) ;
#129579=ORIENTED_EDGE ( 'NONE', *, *, #40904, .T. ) ;
#129580=ORIENTED_EDGE ( 'NONE', *, *, #35816, .T. ) ;
#129581=CARTESIAN_POINT ( 'NONE',  ( 5.599999999999931255, 2.500000000000000000, 3.883716857408420431 ) ) ;
#129582=CARTESIAN_POINT ( 'NONE',  ( 8.749999999999920064, 2.500000000000000000, 5.702370205355745014 ) ) ;
#129583=DIRECTION ( 'NONE',  ( -0.000000000000000000, -1.000000000000000000, -0.000000000000000000 ) ) ;
#129584=AXIS2_PLACEMENT_3D ( 'NONE', #101059, #90586, #40878 ) ;
#129585=AXIS2_PLACEMENT_3D ( 'NONE', #16805, #126798, #107797 ) ;
#129586=EDGE_LOOP ( 'NONE', ( #45447, #107380 ) ) ;
#129587=DIRECTION ( 'NONE',  ( 0.000000000000000000, -0.000000000000000000, 1.000000000000000000 ) ) ;
#129588=CARTESIAN_POINT ( 'NONE',  ( 21.24754738303276724, -0.7337760880902383098, -4.182111650399352953 ) ) ;
#129589=PLANE ( 'NONE',  #369 ) ;
#129590=LINE ( 'NONE', #30743, #44237 ) ;
#129591=AXIS2_PLACEMENT_3D ( 'NONE', #101826, #59345, #9578 ) ;
#129592=AXIS2_PLACEMENT_3D ( 'NONE', #115288, #25641, #65572 ) ;
#129593=ORIENTED_EDGE ( 'NONE', *, *, #1694, .F. ) ;
#129594=LINE ( 'NONE', #39289, #12340 ) ;
#129595=EDGE_CURVE ( 'NONE', #33637, #62109, #68581, .T. ) ;
#129596=ORIENTED_EDGE ( 'NONE', *, *, #80926, .F. ) ;
#129598=DIRECTION ( 'NONE',  ( 0.000000000000000000, -0.000000000000000000, 1.000000000000000000 ) ) ;
#129599=CARTESIAN_POINT ( 'NONE',  ( 13.54999999999990123, 12.50000000000000000, 1.883746621131358934 ) ) ;
#129600=FACE_BOUND ( 'NONE', #13872, .T. ) ;
#129601=VECTOR ( 'NONE', #64863, 1000.000000000000000 ) ;
#129602=CARTESIAN_POINT ( 'NONE',  ( -8.749999999999975131, 2.500000000000000000, -2.065063509461102065 ) ) ;
#129603=CARTESIAN_POINT ( 'NONE',  ( 11.44999999999990692, 2.500000000000000000, 1.718653347947321386 ) ) ;
#129604=CARTESIAN_POINT ( 'NONE',  ( 5.449999999999937117, 12.50000000000000000, -6.495190528383302464 ) ) ;
#129605=EDGE_CURVE ( 'NONE', #118548, #56615, #81123, .T. ) ;
#129606=AXIS2_PLACEMENT_3D ( 'NONE', #98301, #48580, #10560 ) ;
#129607=DIRECTION ( 'NONE',  ( -0.000000000000000000, 1.000000000000000000, -0.000000000000000000 ) ) ;
#129609=DIRECTION ( 'NONE',  ( 0.000000000000000000, 0.000000000000000000, 1.000000000000000000 ) ) ;
#129610=DIRECTION ( 'NONE',  ( 0.000000000000000000, -0.9999939076577903929, 0.003490651415223739937 ) ) ;
#129611=ORIENTED_EDGE ( 'NONE', *, *, #7416, .F. ) ;
#129612=VECTOR ( 'NONE', #54208, 1000.000000000000000 ) ;
#129613=DIRECTION ( 'NONE',  ( 0.000000000000000000, 1.000000000000000000, 0.000000000000000000 ) ) ;
#129614=CARTESIAN_POINT ( 'NONE',  ( 11.64999999999990266, 2.500000000000000000, 2.065063509461097624 ) ) ;
#129615=AXIS2_PLACEMENT_3D ( 'NONE', #63588, #94313, #125077 ) ;
#129616=VERTEX_POINT ( 'NONE', #52536 ) ;
ENDSEC;
END-ISO-10303-21;
